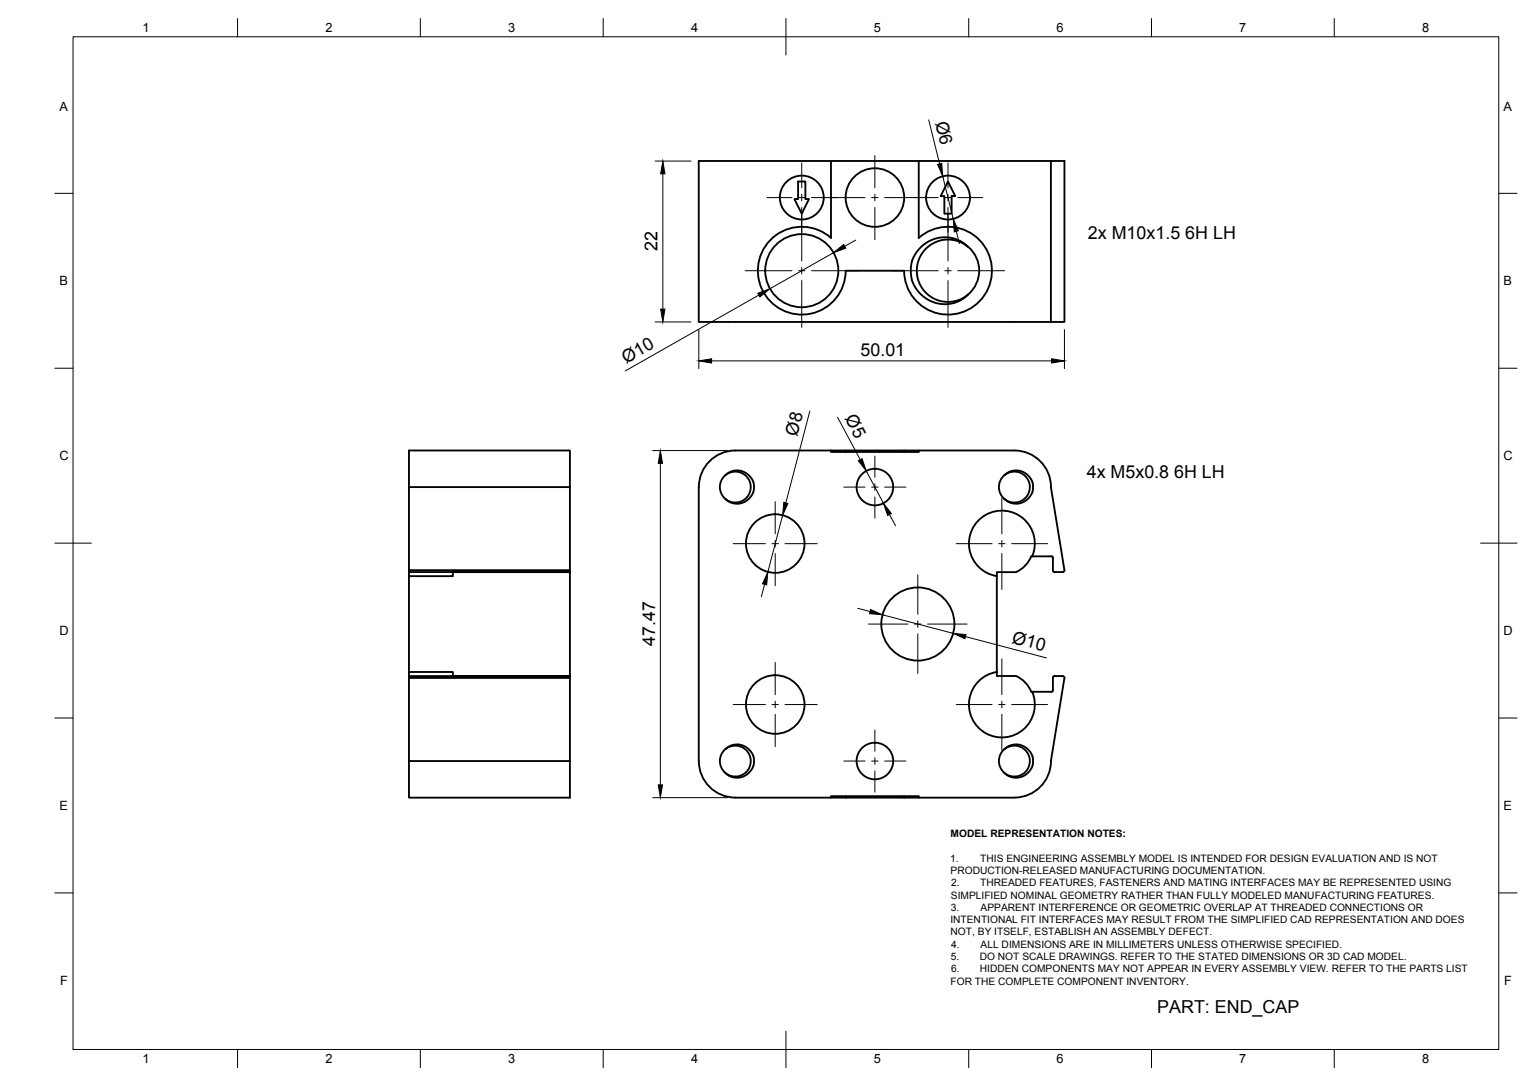
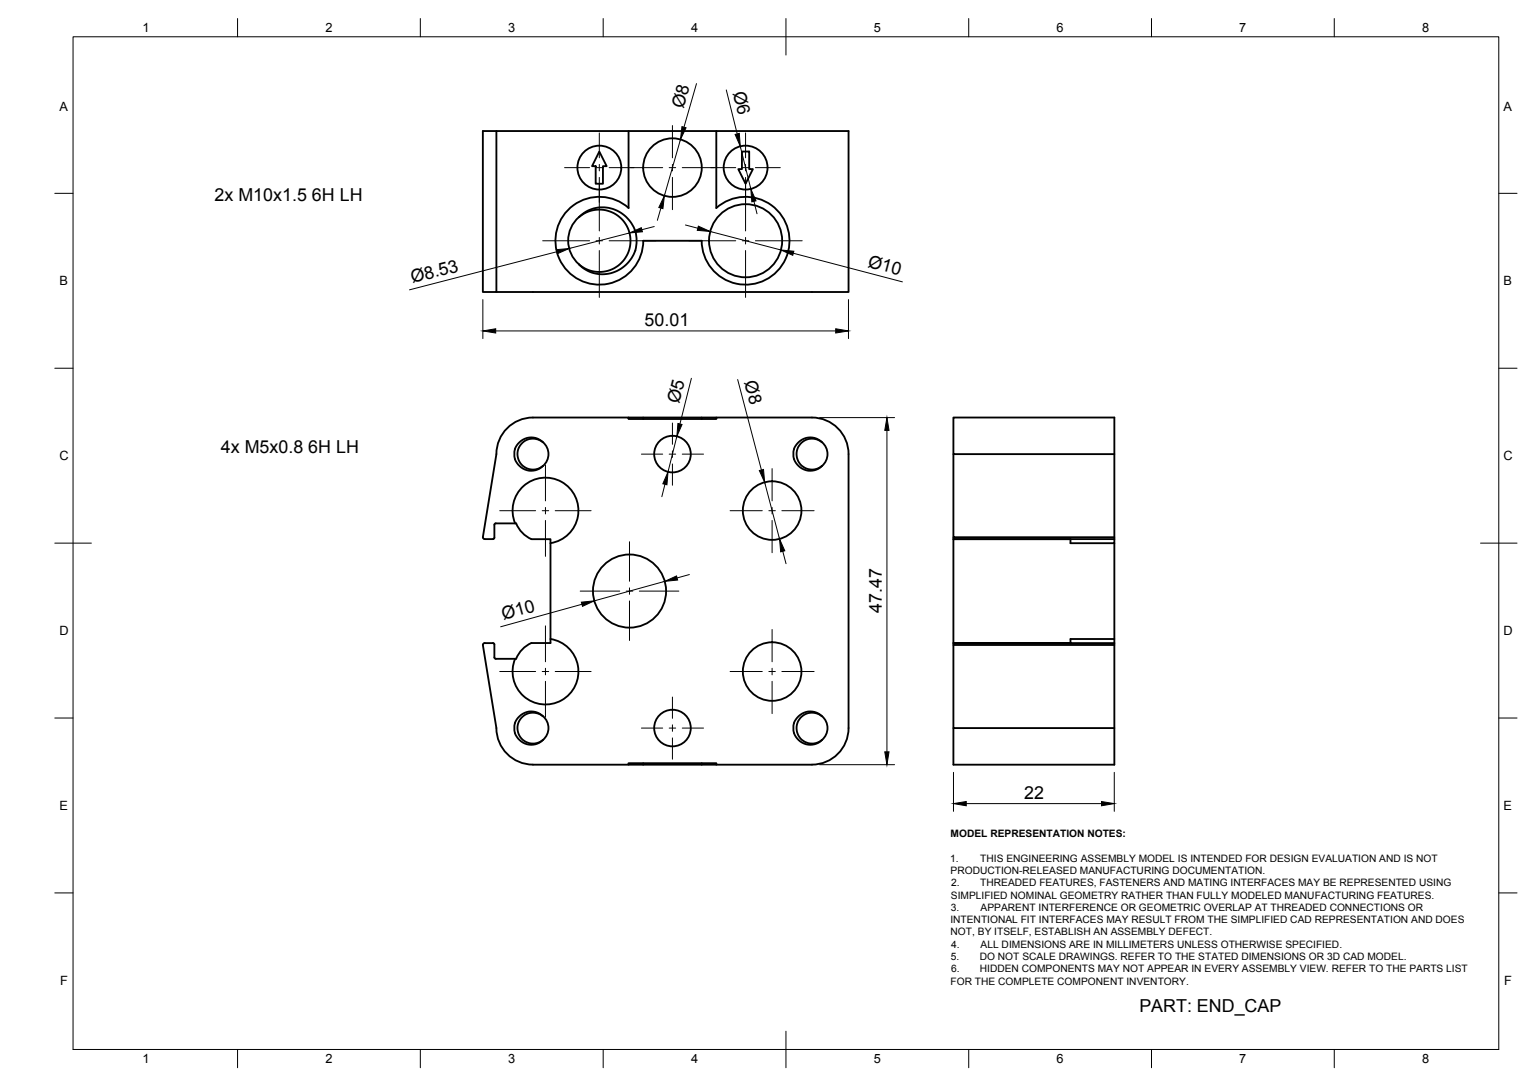
ISO-10303-21;
HEADER;
/* Generated by software containing ST-Developer
 * from STEP Tools, Inc. (www.steptools.com) 
 */

FILE_DESCRIPTION(
/* description */ (''),
/* implementation_level */ '2;1');

FILE_NAME(
/* name */ 'End_Cap.step',
/* time_stamp */ '2026-10-05T11:01:41-07:00',
/* author */ (''),
/* organization */ (''),
/* preprocessor_version */ 'ST-DEVELOPER v20.2',
/* originating_system */ 'Autodesk Translation Framework v15.15.0.0',
/* authorisation */ '');

FILE_SCHEMA (('AUTOMOTIVE_DESIGN { 1 0 10303 214 3 1 1 }'));
ENDSEC;

DATA;
#10=MECHANICAL_DESIGN_GEOMETRIC_PRESENTATION_REPRESENTATION('',(#2139),#215609);
#149=B_SPLINE_SURFACE_WITH_KNOTS('',3,3,((#115948,#115949,#115950,#115951,
#115952,#115953,#115954,#115955,#115956,#115957,#115958,#115959,#115960,
#115961,#115962,#115963,#115964,#115965,#115966,#115967,#115968,#115969,
#115970,#115971,#115972,#115973,#115974,#115975,#115976,#115977,#115978,
#115979,#115980,#115981,#115982,#115983,#115984,#115985,#115986,#115987,
#115988,#115989,#115990,#115991,#115992,#115993,#115994,#115995,#115996,
#115997,#115998,#115999,#116000,#116001),(#116002,#116003,#116004,#116005,
#116006,#116007,#116008,#116009,#116010,#116011,#116012,#116013,#116014,
#116015,#116016,#116017,#116018,#116019,#116020,#116021,#116022,#116023,
#116024,#116025,#116026,#116027,#116028,#116029,#116030,#116031,#116032,
#116033,#116034,#116035,#116036,#116037,#116038,#116039,#116040,#116041,
#116042,#116043,#116044,#116045,#116046,#116047,#116048,#116049,#116050,
#116051,#116052,#116053,#116054,#116055),(#116056,#116057,#116058,#116059,
#116060,#116061,#116062,#116063,#116064,#116065,#116066,#116067,#116068,
#116069,#116070,#116071,#116072,#116073,#116074,#116075,#116076,#116077,
#116078,#116079,#116080,#116081,#116082,#116083,#116084,#116085,#116086,
#116087,#116088,#116089,#116090,#116091,#116092,#116093,#116094,#116095,
#116096,#116097,#116098,#116099,#116100,#116101,#116102,#116103,#116104,
#116105,#116106,#116107,#116108,#116109),(#116110,#116111,#116112,#116113,
#116114,#116115,#116116,#116117,#116118,#116119,#116120,#116121,#116122,
#116123,#116124,#116125,#116126,#116127,#116128,#116129,#116130,#116131,
#116132,#116133,#116134,#116135,#116136,#116137,#116138,#116139,#116140,
#116141,#116142,#116143,#116144,#116145,#116146,#116147,#116148,#116149,
#116150,#116151,#116152,#116153,#116154,#116155,#116156,#116157,#116158,
#116159,#116160,#116161,#116162,#116163)),.UNSPECIFIED.,.F.,.F.,.F.,(4,
4),(4,1,1,1,1,1,1,1,1,1,1,1,1,1,1,1,1,1,1,1,1,1,1,1,1,1,1,1,1,1,1,1,1,1,
1,1,1,1,1,1,1,1,1,1,1,1,1,1,1,1,1,4),(-0.000626221895392836,0.0969365212249631),
(11.8528940954716,12.340290362188,12.8276378599491,13.3149853577101,13.8023328554711,
14.2896803532321,14.7770278509931,15.2643753487541,15.7517228465151,16.2390703442761,
16.7264178420371,17.2137653397981,17.7011128375591,18.1884603353201,18.6758078330811,
19.1631553308421,19.6505028286031,20.1378503263641,20.6251978241251,21.1125453218861,
21.5998928196471,22.0872403174081,22.5745878151691,23.0619353129301,23.5492828106911,
24.5239778062131,25.4986728017351,26.4733677972571,26.9607152950181,27.4480627927791,
27.9354102905401,28.4227577883011,28.9101052860621,29.3974527838231,29.8848002815841,
30.3721477793451,30.8594952771061,31.3468427748671,31.8341902726282,32.3215377703892,
32.8088852681502,33.2962327659112,33.7835802636722,34.2709277614332,34.7582752591942,
35.2456227569552,35.7329702547162,36.2203177524772,36.7076652502382,37.1950127479992,
37.6823602457602,38.1697077435212),.UNSPECIFIED.);
#150=B_SPLINE_SURFACE_WITH_KNOTS('',3,3,((#116370,#116371,#116372,#116373,
#116374,#116375,#116376,#116377,#116378,#116379,#116380,#116381,#116382,
#116383,#116384,#116385,#116386,#116387,#116388,#116389,#116390,#116391,
#116392,#116393,#116394,#116395,#116396,#116397,#116398,#116399,#116400,
#116401,#116402,#116403,#116404,#116405,#116406,#116407,#116408,#116409,
#116410,#116411,#116412,#116413,#116414,#116415,#116416,#116417,#116418,
#116419,#116420,#116421,#116422,#116423),(#116424,#116425,#116426,#116427,
#116428,#116429,#116430,#116431,#116432,#116433,#116434,#116435,#116436,
#116437,#116438,#116439,#116440,#116441,#116442,#116443,#116444,#116445,
#116446,#116447,#116448,#116449,#116450,#116451,#116452,#116453,#116454,
#116455,#116456,#116457,#116458,#116459,#116460,#116461,#116462,#116463,
#116464,#116465,#116466,#116467,#116468,#116469,#116470,#116471,#116472,
#116473,#116474,#116475,#116476,#116477),(#116478,#116479,#116480,#116481,
#116482,#116483,#116484,#116485,#116486,#116487,#116488,#116489,#116490,
#116491,#116492,#116493,#116494,#116495,#116496,#116497,#116498,#116499,
#116500,#116501,#116502,#116503,#116504,#116505,#116506,#116507,#116508,
#116509,#116510,#116511,#116512,#116513,#116514,#116515,#116516,#116517,
#116518,#116519,#116520,#116521,#116522,#116523,#116524,#116525,#116526,
#116527,#116528,#116529,#116530,#116531),(#116532,#116533,#116534,#116535,
#116536,#116537,#116538,#116539,#116540,#116541,#116542,#116543,#116544,
#116545,#116546,#116547,#116548,#116549,#116550,#116551,#116552,#116553,
#116554,#116555,#116556,#116557,#116558,#116559,#116560,#116561,#116562,
#116563,#116564,#116565,#116566,#116567,#116568,#116569,#116570,#116571,
#116572,#116573,#116574,#116575,#116576,#116577,#116578,#116579,#116580,
#116581,#116582,#116583,#116584,#116585)),.UNSPECIFIED.,.F.,.F.,.F.,(4,
4),(4,1,1,1,1,1,1,1,1,1,1,1,1,1,1,1,1,1,1,1,1,1,1,1,1,1,1,1,1,1,1,1,1,1,
1,1,1,1,1,1,1,1,1,1,1,1,1,1,1,1,1,4),(-0.000403511276840155,0.0967757900741628),
(14.399609326548,14.886956824309,15.37430432207,15.861651819831,16.348999317592,
16.836346815353,17.323694313114,17.811041810875,18.298389308636,18.785736806397,
19.273084304158,19.7604318019191,20.2477792996801,20.7351267974411,21.2224742952021,
21.7098217929631,22.1971692907241,22.6845167884851,23.1718642862461,23.6592117840071,
24.1465592817681,24.6339067795291,25.1212542772901,25.6086017750511,26.0959492728121,
27.0706442683341,28.0453392638561,29.0200342593781,29.5073817571391,29.9947292549001,
30.4820767526611,30.9694242504221,31.4567717481831,31.9441192459441,32.4314667437051,
32.9188142414661,33.4061617392271,33.8935092369881,34.3808567347491,34.8682042325101,
35.3555517302711,35.8428992280321,36.3302467257931,36.8175942235541,37.3049417213151,
37.7922892190762,38.2796367168372,38.7669842145982,39.2543317123592,39.7416792101202,
40.2290267078812,40.7164229770097),.UNSPECIFIED.);
#151=B_SPLINE_SURFACE_WITH_KNOTS('',3,3,((#116789,#116790,#116791,#116792,
#116793,#116794,#116795,#116796,#116797,#116798,#116799,#116800,#116801,
#116802,#116803,#116804,#116805,#116806,#116807,#116808,#116809,#116810,
#116811,#116812,#116813,#116814,#116815,#116816,#116817,#116818,#116819,
#116820,#116821,#116822,#116823,#116824,#116825,#116826,#116827,#116828,
#116829,#116830,#116831,#116832,#116833,#116834,#116835,#116836,#116837,
#116838,#116839,#116840,#116841,#116842),(#116843,#116844,#116845,#116846,
#116847,#116848,#116849,#116850,#116851,#116852,#116853,#116854,#116855,
#116856,#116857,#116858,#116859,#116860,#116861,#116862,#116863,#116864,
#116865,#116866,#116867,#116868,#116869,#116870,#116871,#116872,#116873,
#116874,#116875,#116876,#116877,#116878,#116879,#116880,#116881,#116882,
#116883,#116884,#116885,#116886,#116887,#116888,#116889,#116890,#116891,
#116892,#116893,#116894,#116895,#116896),(#116897,#116898,#116899,#116900,
#116901,#116902,#116903,#116904,#116905,#116906,#116907,#116908,#116909,
#116910,#116911,#116912,#116913,#116914,#116915,#116916,#116917,#116918,
#116919,#116920,#116921,#116922,#116923,#116924,#116925,#116926,#116927,
#116928,#116929,#116930,#116931,#116932,#116933,#116934,#116935,#116936,
#116937,#116938,#116939,#116940,#116941,#116942,#116943,#116944,#116945,
#116946,#116947,#116948,#116949,#116950),(#116951,#116952,#116953,#116954,
#116955,#116956,#116957,#116958,#116959,#116960,#116961,#116962,#116963,
#116964,#116965,#116966,#116967,#116968,#116969,#116970,#116971,#116972,
#116973,#116974,#116975,#116976,#116977,#116978,#116979,#116980,#116981,
#116982,#116983,#116984,#116985,#116986,#116987,#116988,#116989,#116990,
#116991,#116992,#116993,#116994,#116995,#116996,#116997,#116998,#116999,
#117000,#117001,#117002,#117003,#117004)),.UNSPECIFIED.,.F.,.F.,.F.,(4,
4),(4,1,1,1,1,1,1,1,1,1,1,1,1,1,1,1,1,1,1,1,1,1,1,1,1,1,1,1,1,1,1,1,1,1,
1,1,1,1,1,1,1,1,1,1,1,1,1,1,1,1,1,4),(-0.000626380093345518,0.0969365193294648),
(11.8528940858174,12.340290362188,12.827637859949,13.31498535771,13.802332855471,
14.289680353232,14.777027850993,15.264375348754,15.751722846515,16.239070344276,
16.7264178420371,17.2137653397981,17.7011128375591,18.1884603353201,18.6758078330811,
19.1631553308421,19.6505028286031,20.1378503263641,20.6251978241251,21.1125453218861,
21.5998928196471,22.0872403174081,22.5745878151691,23.0619353129301,23.5492828106911,
24.5239778062131,25.4986728017351,26.4733677972571,26.9607152950181,27.4480627927791,
27.9354102905401,28.4227577883011,28.9101052860621,29.3974527838231,29.8848002815841,
30.3721477793451,30.8594952771061,31.3468427748671,31.8341902726281,32.3215377703891,
32.8088852681501,33.2962327659111,33.7835802636721,34.2709277614331,34.7582752591941,
35.2456227569552,35.7329702547162,36.2203177524772,36.7076652502382,37.1950127479992,
37.6823602457602,38.1697077435212),.UNSPECIFIED.);
#152=B_SPLINE_SURFACE_WITH_KNOTS('',3,3,((#117214,#117215,#117216,#117217,
#117218,#117219,#117220,#117221,#117222,#117223,#117224,#117225,#117226,
#117227,#117228,#117229,#117230,#117231,#117232,#117233,#117234,#117235,
#117236,#117237,#117238,#117239,#117240,#117241,#117242,#117243,#117244,
#117245,#117246,#117247,#117248,#117249,#117250,#117251,#117252,#117253,
#117254,#117255,#117256,#117257,#117258,#117259,#117260,#117261,#117262,
#117263,#117264,#117265,#117266,#117267),(#117268,#117269,#117270,#117271,
#117272,#117273,#117274,#117275,#117276,#117277,#117278,#117279,#117280,
#117281,#117282,#117283,#117284,#117285,#117286,#117287,#117288,#117289,
#117290,#117291,#117292,#117293,#117294,#117295,#117296,#117297,#117298,
#117299,#117300,#117301,#117302,#117303,#117304,#117305,#117306,#117307,
#117308,#117309,#117310,#117311,#117312,#117313,#117314,#117315,#117316,
#117317,#117318,#117319,#117320,#117321),(#117322,#117323,#117324,#117325,
#117326,#117327,#117328,#117329,#117330,#117331,#117332,#117333,#117334,
#117335,#117336,#117337,#117338,#117339,#117340,#117341,#117342,#117343,
#117344,#117345,#117346,#117347,#117348,#117349,#117350,#117351,#117352,
#117353,#117354,#117355,#117356,#117357,#117358,#117359,#117360,#117361,
#117362,#117363,#117364,#117365,#117366,#117367,#117368,#117369,#117370,
#117371,#117372,#117373,#117374,#117375),(#117376,#117377,#117378,#117379,
#117380,#117381,#117382,#117383,#117384,#117385,#117386,#117387,#117388,
#117389,#117390,#117391,#117392,#117393,#117394,#117395,#117396,#117397,
#117398,#117399,#117400,#117401,#117402,#117403,#117404,#117405,#117406,
#117407,#117408,#117409,#117410,#117411,#117412,#117413,#117414,#117415,
#117416,#117417,#117418,#117419,#117420,#117421,#117422,#117423,#117424,
#117425,#117426,#117427,#117428,#117429)),.UNSPECIFIED.,.F.,.F.,.F.,(4,
4),(4,1,1,1,1,1,1,1,1,1,1,1,1,1,1,1,1,1,1,1,1,1,1,1,1,1,1,1,1,1,1,1,1,1,
1,1,1,1,1,1,1,1,1,1,1,1,1,1,1,1,1,4),(-0.000403508817394493,0.0967757699182735),
(14.399609326548,14.886956824309,15.37430432207,15.861651819831,16.348999317592,
16.836346815353,17.323694313114,17.811041810875,18.298389308636,18.785736806397,
19.273084304158,19.760431801919,20.24777929968,20.735126797441,21.222474295202,
21.709821792963,22.1971692907241,22.6845167884851,23.1718642862461,23.6592117840071,
24.1465592817681,24.6339067795291,25.1212542772901,25.6086017750511,26.0959492728121,
27.0706442683341,28.0453392638561,29.0200342593781,29.5073817571391,29.9947292549001,
30.4820767526611,30.9694242504221,31.4567717481831,31.9441192459441,32.4314667437051,
32.9188142414661,33.4061617392271,33.8935092369881,34.3808567347491,34.8682042325101,
35.3555517302711,35.8428992280321,36.3302467257931,36.8175942235541,37.3049417213151,
37.7922892190761,38.2796367168371,38.7669842145981,39.2543317123591,39.7416792101202,
40.2290267078812,40.7164229892059),.UNSPECIFIED.);
#153=B_SPLINE_SURFACE_WITH_KNOTS('',3,3,((#117642,#117643,#117644,#117645,
#117646,#117647,#117648,#117649,#117650,#117651,#117652,#117653,#117654,
#117655,#117656,#117657,#117658,#117659,#117660,#117661,#117662,#117663,
#117664,#117665,#117666,#117667,#117668,#117669,#117670,#117671,#117672,
#117673,#117674,#117675,#117676,#117677,#117678,#117679,#117680,#117681,
#117682,#117683,#117684,#117685,#117686,#117687,#117688,#117689,#117690,
#117691,#117692,#117693,#117694,#117695,#117696,#117697,#117698,#117699,
#117700,#117701,#117702,#117703,#117704,#117705,#117706,#117707,#117708,
#117709,#117710,#117711,#117712,#117713,#117714,#117715,#117716,#117717,
#117718,#117719,#117720,#117721,#117722,#117723,#117724,#117725,#117726,
#117727,#117728,#117729,#117730,#117731,#117732,#117733,#117734,#117735,
#117736,#117737,#117738,#117739,#117740,#117741,#117742,#117743,#117744,
#117745,#117746,#117747,#117748,#117749,#117750,#117751,#117752,#117753,
#117754,#117755,#117756,#117757,#117758,#117759,#117760,#117761,#117762,
#117763,#117764,#117765,#117766,#117767,#117768,#117769,#117770,#117771,
#117772,#117773,#117774,#117775,#117776,#117777,#117778,#117779,#117780,
#117781,#117782,#117783,#117784,#117785,#117786,#117787,#117788,#117789,
#117790,#117791,#117792,#117793,#117794,#117795,#117796,#117797,#117798,
#117799,#117800,#117801,#117802,#117803,#117804,#117805,#117806,#117807,
#117808,#117809,#117810,#117811,#117812,#117813,#117814,#117815,#117816,
#117817,#117818,#117819),(#117820,#117821,#117822,#117823,#117824,#117825,
#117826,#117827,#117828,#117829,#117830,#117831,#117832,#117833,#117834,
#117835,#117836,#117837,#117838,#117839,#117840,#117841,#117842,#117843,
#117844,#117845,#117846,#117847,#117848,#117849,#117850,#117851,#117852,
#117853,#117854,#117855,#117856,#117857,#117858,#117859,#117860,#117861,
#117862,#117863,#117864,#117865,#117866,#117867,#117868,#117869,#117870,
#117871,#117872,#117873,#117874,#117875,#117876,#117877,#117878,#117879,
#117880,#117881,#117882,#117883,#117884,#117885,#117886,#117887,#117888,
#117889,#117890,#117891,#117892,#117893,#117894,#117895,#117896,#117897,
#117898,#117899,#117900,#117901,#117902,#117903,#117904,#117905,#117906,
#117907,#117908,#117909,#117910,#117911,#117912,#117913,#117914,#117915,
#117916,#117917,#117918,#117919,#117920,#117921,#117922,#117923,#117924,
#117925,#117926,#117927,#117928,#117929,#117930,#117931,#117932,#117933,
#117934,#117935,#117936,#117937,#117938,#117939,#117940,#117941,#117942,
#117943,#117944,#117945,#117946,#117947,#117948,#117949,#117950,#117951,
#117952,#117953,#117954,#117955,#117956,#117957,#117958,#117959,#117960,
#117961,#117962,#117963,#117964,#117965,#117966,#117967,#117968,#117969,
#117970,#117971,#117972,#117973,#117974,#117975,#117976,#117977,#117978,
#117979,#117980,#117981,#117982,#117983,#117984,#117985,#117986,#117987,
#117988,#117989,#117990,#117991,#117992,#117993,#117994,#117995,#117996,
#117997),(#117998,#117999,#118000,#118001,#118002,#118003,#118004,#118005,
#118006,#118007,#118008,#118009,#118010,#118011,#118012,#118013,#118014,
#118015,#118016,#118017,#118018,#118019,#118020,#118021,#118022,#118023,
#118024,#118025,#118026,#118027,#118028,#118029,#118030,#118031,#118032,
#118033,#118034,#118035,#118036,#118037,#118038,#118039,#118040,#118041,
#118042,#118043,#118044,#118045,#118046,#118047,#118048,#118049,#118050,
#118051,#118052,#118053,#118054,#118055,#118056,#118057,#118058,#118059,
#118060,#118061,#118062,#118063,#118064,#118065,#118066,#118067,#118068,
#118069,#118070,#118071,#118072,#118073,#118074,#118075,#118076,#118077,
#118078,#118079,#118080,#118081,#118082,#118083,#118084,#118085,#118086,
#118087,#118088,#118089,#118090,#118091,#118092,#118093,#118094,#118095,
#118096,#118097,#118098,#118099,#118100,#118101,#118102,#118103,#118104,
#118105,#118106,#118107,#118108,#118109,#118110,#118111,#118112,#118113,
#118114,#118115,#118116,#118117,#118118,#118119,#118120,#118121,#118122,
#118123,#118124,#118125,#118126,#118127,#118128,#118129,#118130,#118131,
#118132,#118133,#118134,#118135,#118136,#118137,#118138,#118139,#118140,
#118141,#118142,#118143,#118144,#118145,#118146,#118147,#118148,#118149,
#118150,#118151,#118152,#118153,#118154,#118155,#118156,#118157,#118158,
#118159,#118160,#118161,#118162,#118163,#118164,#118165,#118166,#118167,
#118168,#118169,#118170,#118171,#118172,#118173,#118174,#118175),(#118176,
#118177,#118178,#118179,#118180,#118181,#118182,#118183,#118184,#118185,
#118186,#118187,#118188,#118189,#118190,#118191,#118192,#118193,#118194,
#118195,#118196,#118197,#118198,#118199,#118200,#118201,#118202,#118203,
#118204,#118205,#118206,#118207,#118208,#118209,#118210,#118211,#118212,
#118213,#118214,#118215,#118216,#118217,#118218,#118219,#118220,#118221,
#118222,#118223,#118224,#118225,#118226,#118227,#118228,#118229,#118230,
#118231,#118232,#118233,#118234,#118235,#118236,#118237,#118238,#118239,
#118240,#118241,#118242,#118243,#118244,#118245,#118246,#118247,#118248,
#118249,#118250,#118251,#118252,#118253,#118254,#118255,#118256,#118257,
#118258,#118259,#118260,#118261,#118262,#118263,#118264,#118265,#118266,
#118267,#118268,#118269,#118270,#118271,#118272,#118273,#118274,#118275,
#118276,#118277,#118278,#118279,#118280,#118281,#118282,#118283,#118284,
#118285,#118286,#118287,#118288,#118289,#118290,#118291,#118292,#118293,
#118294,#118295,#118296,#118297,#118298,#118299,#118300,#118301,#118302,
#118303,#118304,#118305,#118306,#118307,#118308,#118309,#118310,#118311,
#118312,#118313,#118314,#118315,#118316,#118317,#118318,#118319,#118320,
#118321,#118322,#118323,#118324,#118325,#118326,#118327,#118328,#118329,
#118330,#118331,#118332,#118333,#118334,#118335,#118336,#118337,#118338,
#118339,#118340,#118341,#118342,#118343,#118344,#118345,#118346,#118347,
#118348,#118349,#118350,#118351,#118352,#118353)),.UNSPECIFIED.,.F.,.F.,
 .F.,(4,4),(4,1,1,1,1,1,1,1,1,1,1,1,1,1,1,1,1,1,1,1,1,1,1,1,1,1,1,1,1,1,
1,1,1,1,1,1,1,1,1,1,1,1,1,1,1,1,1,1,1,1,1,1,1,1,1,1,1,1,1,1,1,1,1,1,1,1,
1,1,1,1,1,1,1,1,1,1,1,1,1,1,1,1,1,1,1,1,1,1,1,1,1,1,1,1,1,1,1,1,1,1,1,1,
1,1,1,1,1,1,1,1,1,1,1,1,1,1,1,1,1,1,1,1,1,1,1,1,1,1,1,1,1,1,1,1,1,1,1,1,
1,1,1,1,1,1,1,1,1,1,1,1,1,1,1,1,1,1,1,1,1,1,1,1,1,1,1,1,1,1,1,1,1,1,1,1,
1,4),(-0.000439606948779746,0.0515314320759051),(11.8664846275776,12.8657606844883,
13.8645971344502,14.8634335844121,15.8622700343739,16.8611064843358,17.8599429342977,
18.8587793842595,19.8576158342214,20.8564522841833,21.8552887341452,22.854125184107,
23.8529616340689,24.8517980840308,25.8506345339927,26.8494709839545,27.8483074339164,
28.8471438838783,29.8459803338402,30.844816783802,31.8436532337639,32.8424896837258,
33.8413261336877,34.8401625836495,35.8389990336114,36.8378354835733,37.8366719335352,
38.835508383497,39.8343448334589,40.8331812834208,41.8320177333826,42.8308541833445,
43.8296906333064,44.8285270832683,45.8273635332301,46.826199983192,47.8250364331539,
48.8238728831158,49.8227093330776,50.8215457830395,51.8203822330014,52.8192186829633,
53.8180551329251,54.816891582887,55.8157280328489,56.8145644828108,57.8134009327726,
58.8122373827345,59.8110738326964,60.8099102826583,61.8087467326201,62.807583182582,
63.8064196325439,64.8052560825058,65.8040925324676,66.8029289824295,67.8017654323914,
68.8006018823532,69.7994383323151,70.798274782277,71.7971112322389,72.7959476822007,
73.7947841321626,74.7936205821245,75.7924570320864,76.7912934820482,77.7901299320101,
78.788966381972,79.7878028319339,80.7866392818957,81.7854757318576,82.7843121818195,
83.7831486317814,84.7819850817432,85.7808215317051,86.779657981667,87.7784944316288,
88.7773308815907,89.7761673315526,90.7750037815145,91.7738402314764,92.7726766814382,
93.7715131314001,94.770349581362,95.7691860313238,96.7680224812857,97.7668589312476,
98.7656953812095,99.7645318311714,100.763368281133,101.762204731095,102.761041181057,
103.759877631019,104.758714080981,105.757550530943,106.756386980904,107.755223430866,
108.754059880828,109.75289633079,110.751732780752,111.750569230714,112.749405680676,
113.748242130638,114.747078580599,115.745915030561,116.744751480523,117.743587930485,
118.742424380447,119.741260830409,120.740097280371,121.738933730333,122.737770180294,
123.736606630256,124.735443080218,125.73427953018,126.733115980142,127.731952430104,
128.730788880066,129.729625330028,130.728461779989,131.727298229951,132.726134679913,
133.724971129875,134.723807579837,135.722644029799,136.721480479761,137.720316929723,
138.719153379684,139.717989829646,140.716826279608,141.71566272957,142.714499179532,
143.713335629494,144.712172079456,145.711008529418,146.709844979379,147.708681429341,
148.707517879303,149.706354329265,150.705190779227,151.704027229189,152.702863679151,
153.701700129113,154.700536579074,155.699373029036,156.698209478998,157.69704592896,
158.695882378922,159.694718828884,160.693555278846,161.692391728808,162.691228178769,
163.690064628731,164.688901078693,165.687737528655,166.686573978617,167.685410428579,
168.684246878541,169.683083328503,170.681919778464,171.680756228426,172.679592678388,
173.67842912835,174.677265578312,175.676102028274,176.674938478236,177.673774928198,
178.672611378159,179.671447828121,180.670284278083,181.669120728045,182.667957178007,
183.666793627969,184.665630077931,185.664466527893,186.663302977854),
 .UNSPECIFIED.);
#154=B_SPLINE_SURFACE_WITH_KNOTS('',3,3,((#118442,#118443,#118444,#118445,
#118446,#118447,#118448,#118449,#118450,#118451,#118452,#118453,#118454,
#118455,#118456,#118457,#118458,#118459,#118460,#118461,#118462,#118463,
#118464,#118465,#118466,#118467,#118468,#118469,#118470,#118471,#118472,
#118473,#118474,#118475,#118476,#118477,#118478,#118479,#118480,#118481,
#118482,#118483,#118484,#118485,#118486,#118487,#118488,#118489,#118490,
#118491,#118492,#118493,#118494,#118495,#118496,#118497,#118498,#118499,
#118500,#118501,#118502,#118503,#118504,#118505,#118506,#118507,#118508,
#118509,#118510,#118511,#118512,#118513,#118514,#118515,#118516,#118517,
#118518,#118519,#118520,#118521,#118522,#118523,#118524,#118525,#118526,
#118527,#118528,#118529,#118530,#118531,#118532,#118533,#118534,#118535,
#118536,#118537,#118538,#118539,#118540,#118541,#118542,#118543,#118544,
#118545,#118546,#118547,#118548,#118549,#118550,#118551,#118552,#118553,
#118554,#118555,#118556,#118557,#118558,#118559,#118560,#118561,#118562,
#118563,#118564,#118565,#118566,#118567,#118568,#118569,#118570,#118571,
#118572,#118573,#118574,#118575,#118576,#118577,#118578,#118579,#118580,
#118581,#118582,#118583,#118584,#118585,#118586,#118587,#118588,#118589,
#118590,#118591,#118592,#118593,#118594,#118595,#118596,#118597,#118598,
#118599,#118600,#118601,#118602,#118603,#118604,#118605,#118606,#118607,
#118608,#118609,#118610,#118611,#118612,#118613,#118614,#118615,#118616,
#118617,#118618,#118619),(#118620,#118621,#118622,#118623,#118624,#118625,
#118626,#118627,#118628,#118629,#118630,#118631,#118632,#118633,#118634,
#118635,#118636,#118637,#118638,#118639,#118640,#118641,#118642,#118643,
#118644,#118645,#118646,#118647,#118648,#118649,#118650,#118651,#118652,
#118653,#118654,#118655,#118656,#118657,#118658,#118659,#118660,#118661,
#118662,#118663,#118664,#118665,#118666,#118667,#118668,#118669,#118670,
#118671,#118672,#118673,#118674,#118675,#118676,#118677,#118678,#118679,
#118680,#118681,#118682,#118683,#118684,#118685,#118686,#118687,#118688,
#118689,#118690,#118691,#118692,#118693,#118694,#118695,#118696,#118697,
#118698,#118699,#118700,#118701,#118702,#118703,#118704,#118705,#118706,
#118707,#118708,#118709,#118710,#118711,#118712,#118713,#118714,#118715,
#118716,#118717,#118718,#118719,#118720,#118721,#118722,#118723,#118724,
#118725,#118726,#118727,#118728,#118729,#118730,#118731,#118732,#118733,
#118734,#118735,#118736,#118737,#118738,#118739,#118740,#118741,#118742,
#118743,#118744,#118745,#118746,#118747,#118748,#118749,#118750,#118751,
#118752,#118753,#118754,#118755,#118756,#118757,#118758,#118759,#118760,
#118761,#118762,#118763,#118764,#118765,#118766,#118767,#118768,#118769,
#118770,#118771,#118772,#118773,#118774,#118775,#118776,#118777,#118778,
#118779,#118780,#118781,#118782,#118783,#118784,#118785,#118786,#118787,
#118788,#118789,#118790,#118791,#118792,#118793,#118794,#118795,#118796,
#118797),(#118798,#118799,#118800,#118801,#118802,#118803,#118804,#118805,
#118806,#118807,#118808,#118809,#118810,#118811,#118812,#118813,#118814,
#118815,#118816,#118817,#118818,#118819,#118820,#118821,#118822,#118823,
#118824,#118825,#118826,#118827,#118828,#118829,#118830,#118831,#118832,
#118833,#118834,#118835,#118836,#118837,#118838,#118839,#118840,#118841,
#118842,#118843,#118844,#118845,#118846,#118847,#118848,#118849,#118850,
#118851,#118852,#118853,#118854,#118855,#118856,#118857,#118858,#118859,
#118860,#118861,#118862,#118863,#118864,#118865,#118866,#118867,#118868,
#118869,#118870,#118871,#118872,#118873,#118874,#118875,#118876,#118877,
#118878,#118879,#118880,#118881,#118882,#118883,#118884,#118885,#118886,
#118887,#118888,#118889,#118890,#118891,#118892,#118893,#118894,#118895,
#118896,#118897,#118898,#118899,#118900,#118901,#118902,#118903,#118904,
#118905,#118906,#118907,#118908,#118909,#118910,#118911,#118912,#118913,
#118914,#118915,#118916,#118917,#118918,#118919,#118920,#118921,#118922,
#118923,#118924,#118925,#118926,#118927,#118928,#118929,#118930,#118931,
#118932,#118933,#118934,#118935,#118936,#118937,#118938,#118939,#118940,
#118941,#118942,#118943,#118944,#118945,#118946,#118947,#118948,#118949,
#118950,#118951,#118952,#118953,#118954,#118955,#118956,#118957,#118958,
#118959,#118960,#118961,#118962,#118963,#118964,#118965,#118966,#118967,
#118968,#118969,#118970,#118971,#118972,#118973,#118974,#118975),(#118976,
#118977,#118978,#118979,#118980,#118981,#118982,#118983,#118984,#118985,
#118986,#118987,#118988,#118989,#118990,#118991,#118992,#118993,#118994,
#118995,#118996,#118997,#118998,#118999,#119000,#119001,#119002,#119003,
#119004,#119005,#119006,#119007,#119008,#119009,#119010,#119011,#119012,
#119013,#119014,#119015,#119016,#119017,#119018,#119019,#119020,#119021,
#119022,#119023,#119024,#119025,#119026,#119027,#119028,#119029,#119030,
#119031,#119032,#119033,#119034,#119035,#119036,#119037,#119038,#119039,
#119040,#119041,#119042,#119043,#119044,#119045,#119046,#119047,#119048,
#119049,#119050,#119051,#119052,#119053,#119054,#119055,#119056,#119057,
#119058,#119059,#119060,#119061,#119062,#119063,#119064,#119065,#119066,
#119067,#119068,#119069,#119070,#119071,#119072,#119073,#119074,#119075,
#119076,#119077,#119078,#119079,#119080,#119081,#119082,#119083,#119084,
#119085,#119086,#119087,#119088,#119089,#119090,#119091,#119092,#119093,
#119094,#119095,#119096,#119097,#119098,#119099,#119100,#119101,#119102,
#119103,#119104,#119105,#119106,#119107,#119108,#119109,#119110,#119111,
#119112,#119113,#119114,#119115,#119116,#119117,#119118,#119119,#119120,
#119121,#119122,#119123,#119124,#119125,#119126,#119127,#119128,#119129,
#119130,#119131,#119132,#119133,#119134,#119135,#119136,#119137,#119138,
#119139,#119140,#119141,#119142,#119143,#119144,#119145,#119146,#119147,
#119148,#119149,#119150,#119151,#119152,#119153)),.UNSPECIFIED.,.F.,.F.,
 .F.,(4,4),(4,1,1,1,1,1,1,1,1,1,1,1,1,1,1,1,1,1,1,1,1,1,1,1,1,1,1,1,1,1,
1,1,1,1,1,1,1,1,1,1,1,1,1,1,1,1,1,1,1,1,1,1,1,1,1,1,1,1,1,1,1,1,1,1,1,1,
1,1,1,1,1,1,1,1,1,1,1,1,1,1,1,1,1,1,1,1,1,1,1,1,1,1,1,1,1,1,1,1,1,1,1,1,
1,1,1,1,1,1,1,1,1,1,1,1,1,1,1,1,1,1,1,1,1,1,1,1,1,1,1,1,1,1,1,1,1,1,1,1,
1,1,1,1,1,1,1,1,1,1,1,1,1,1,1,1,1,1,1,1,1,1,1,1,1,1,1,1,1,1,1,1,1,1,1,1,
1,4),(-0.000378201108639058,0.051592837406338),(14.3986268518925,15.3974633018543,
16.3962997518162,17.3951362017781,18.39397265174,19.3928091017018,20.3916455516637,
21.3904820016256,22.3893184515875,23.3881549015493,24.3869913515112,25.3858278014731,
26.3846642514349,27.3835007013968,28.3823371513587,29.3811736013206,30.3800100512824,
31.3788465012443,32.3776829512062,33.3765194011681,34.3753558511299,35.3741923010918,
36.3730287510537,37.3718652010156,38.3707016509774,39.3695381009393,40.3683745509012,
41.3672110008631,42.3660474508249,43.3648839007868,44.3637203507487,45.3625568007106,
46.3613932506724,47.3602297006343,48.3590661505962,49.3579026005581,50.3567390505199,
51.3555755004818,52.3544119504437,53.3532484004055,54.3520848503674,55.3509213003293,
56.3497577502912,57.348594200253,58.3474306502149,59.3462671001768,60.3451035501387,
61.3439400001005,62.3427764500624,63.3416129000243,64.3404493499862,65.339285799948,
66.3381222499099,67.3369586998718,68.3357951498337,69.3346315997955,70.3334680497574,
71.3323044997193,72.3311409496812,73.329977399643,74.3288138496049,75.3276502995668,
76.3264867495287,77.3253231994905,78.3241596494524,79.3229960994143,80.3218325493762,
81.320668999338,82.3195054492999,83.3183418992618,84.3171783492237,85.3160147991855,
86.3148512491474,87.3136876991093,88.3125241490712,89.311360599033,90.3101970489949,
91.3090334989568,92.3078699489186,93.3067063988805,94.3055428488424,95.3043792988043,
96.3032157487661,97.302052198728,98.3008886486899,99.2997250986518,100.298561548614,
101.297397998576,102.296234448537,103.295070898499,104.293907348461,105.292743798423,
106.291580248385,107.290416698347,108.289253148309,109.288089598271,110.286926048232,
111.285762498194,112.284598948156,113.283435398118,114.28227184808,115.281108298042,
116.279944748004,117.278781197966,118.277617647927,119.276454097889,120.275290547851,
121.274126997813,122.272963447775,123.271799897737,124.270636347699,125.26947279766,
126.268309247622,127.267145697584,128.265982147546,129.264818597508,130.26365504747,
131.262491497432,132.261327947394,133.260164397355,134.259000847317,135.257837297279,
136.256673747241,137.255510197203,138.254346647165,139.253183097127,140.252019547089,
141.25085599705,142.249692447012,143.248528896974,144.247365346936,145.246201796898,
146.24503824686,147.243874696822,148.242711146784,149.241547596745,150.240384046707,
151.239220496669,152.238056946631,153.236893396593,154.235729846555,155.234566296517,
156.233402746479,157.23223919644,158.231075646402,159.229912096364,160.228748546326,
161.227584996288,162.22642144625,163.225257896212,164.224094346174,165.222930796135,
166.221767246097,167.220603696059,168.219440146021,169.218276595983,170.217113045945,
171.215949495907,172.214785945869,173.21362239583,174.212458845792,175.211295295754,
176.210131745716,177.208968195678,178.20780464564,179.206641095602,180.205477545564,
181.204313995525,182.203150445487,183.201986895449,184.200823345411,185.199659795373,
186.198496245335,187.197332695297,188.196169145259,189.195445198776),
 .UNSPECIFIED.);
#155=B_SPLINE_SURFACE_WITH_KNOTS('',3,3,((#119245,#119246,#119247,#119248,
#119249,#119250,#119251,#119252,#119253,#119254,#119255,#119256,#119257,
#119258,#119259,#119260,#119261,#119262,#119263,#119264,#119265,#119266,
#119267,#119268,#119269,#119270,#119271,#119272,#119273,#119274,#119275,
#119276,#119277,#119278,#119279,#119280,#119281,#119282,#119283,#119284,
#119285,#119286,#119287,#119288,#119289,#119290,#119291,#119292,#119293,
#119294,#119295,#119296,#119297,#119298,#119299,#119300,#119301,#119302,
#119303,#119304,#119305,#119306,#119307,#119308,#119309,#119310,#119311,
#119312,#119313,#119314,#119315,#119316,#119317,#119318,#119319,#119320,
#119321,#119322,#119323,#119324,#119325,#119326,#119327,#119328,#119329,
#119330,#119331,#119332,#119333,#119334,#119335,#119336,#119337,#119338,
#119339,#119340,#119341,#119342,#119343,#119344,#119345,#119346,#119347,
#119348,#119349,#119350,#119351,#119352,#119353,#119354,#119355,#119356,
#119357,#119358,#119359,#119360,#119361,#119362,#119363,#119364,#119365,
#119366,#119367,#119368,#119369,#119370,#119371,#119372,#119373,#119374,
#119375,#119376,#119377,#119378,#119379,#119380,#119381,#119382,#119383,
#119384,#119385,#119386,#119387,#119388,#119389,#119390,#119391,#119392,
#119393,#119394,#119395,#119396,#119397,#119398,#119399,#119400,#119401,
#119402,#119403,#119404,#119405,#119406,#119407,#119408,#119409,#119410,
#119411,#119412,#119413,#119414,#119415,#119416,#119417,#119418,#119419,
#119420,#119421,#119422),(#119423,#119424,#119425,#119426,#119427,#119428,
#119429,#119430,#119431,#119432,#119433,#119434,#119435,#119436,#119437,
#119438,#119439,#119440,#119441,#119442,#119443,#119444,#119445,#119446,
#119447,#119448,#119449,#119450,#119451,#119452,#119453,#119454,#119455,
#119456,#119457,#119458,#119459,#119460,#119461,#119462,#119463,#119464,
#119465,#119466,#119467,#119468,#119469,#119470,#119471,#119472,#119473,
#119474,#119475,#119476,#119477,#119478,#119479,#119480,#119481,#119482,
#119483,#119484,#119485,#119486,#119487,#119488,#119489,#119490,#119491,
#119492,#119493,#119494,#119495,#119496,#119497,#119498,#119499,#119500,
#119501,#119502,#119503,#119504,#119505,#119506,#119507,#119508,#119509,
#119510,#119511,#119512,#119513,#119514,#119515,#119516,#119517,#119518,
#119519,#119520,#119521,#119522,#119523,#119524,#119525,#119526,#119527,
#119528,#119529,#119530,#119531,#119532,#119533,#119534,#119535,#119536,
#119537,#119538,#119539,#119540,#119541,#119542,#119543,#119544,#119545,
#119546,#119547,#119548,#119549,#119550,#119551,#119552,#119553,#119554,
#119555,#119556,#119557,#119558,#119559,#119560,#119561,#119562,#119563,
#119564,#119565,#119566,#119567,#119568,#119569,#119570,#119571,#119572,
#119573,#119574,#119575,#119576,#119577,#119578,#119579,#119580,#119581,
#119582,#119583,#119584,#119585,#119586,#119587,#119588,#119589,#119590,
#119591,#119592,#119593,#119594,#119595,#119596,#119597,#119598,#119599,
#119600),(#119601,#119602,#119603,#119604,#119605,#119606,#119607,#119608,
#119609,#119610,#119611,#119612,#119613,#119614,#119615,#119616,#119617,
#119618,#119619,#119620,#119621,#119622,#119623,#119624,#119625,#119626,
#119627,#119628,#119629,#119630,#119631,#119632,#119633,#119634,#119635,
#119636,#119637,#119638,#119639,#119640,#119641,#119642,#119643,#119644,
#119645,#119646,#119647,#119648,#119649,#119650,#119651,#119652,#119653,
#119654,#119655,#119656,#119657,#119658,#119659,#119660,#119661,#119662,
#119663,#119664,#119665,#119666,#119667,#119668,#119669,#119670,#119671,
#119672,#119673,#119674,#119675,#119676,#119677,#119678,#119679,#119680,
#119681,#119682,#119683,#119684,#119685,#119686,#119687,#119688,#119689,
#119690,#119691,#119692,#119693,#119694,#119695,#119696,#119697,#119698,
#119699,#119700,#119701,#119702,#119703,#119704,#119705,#119706,#119707,
#119708,#119709,#119710,#119711,#119712,#119713,#119714,#119715,#119716,
#119717,#119718,#119719,#119720,#119721,#119722,#119723,#119724,#119725,
#119726,#119727,#119728,#119729,#119730,#119731,#119732,#119733,#119734,
#119735,#119736,#119737,#119738,#119739,#119740,#119741,#119742,#119743,
#119744,#119745,#119746,#119747,#119748,#119749,#119750,#119751,#119752,
#119753,#119754,#119755,#119756,#119757,#119758,#119759,#119760,#119761,
#119762,#119763,#119764,#119765,#119766,#119767,#119768,#119769,#119770,
#119771,#119772,#119773,#119774,#119775,#119776,#119777,#119778),(#119779,
#119780,#119781,#119782,#119783,#119784,#119785,#119786,#119787,#119788,
#119789,#119790,#119791,#119792,#119793,#119794,#119795,#119796,#119797,
#119798,#119799,#119800,#119801,#119802,#119803,#119804,#119805,#119806,
#119807,#119808,#119809,#119810,#119811,#119812,#119813,#119814,#119815,
#119816,#119817,#119818,#119819,#119820,#119821,#119822,#119823,#119824,
#119825,#119826,#119827,#119828,#119829,#119830,#119831,#119832,#119833,
#119834,#119835,#119836,#119837,#119838,#119839,#119840,#119841,#119842,
#119843,#119844,#119845,#119846,#119847,#119848,#119849,#119850,#119851,
#119852,#119853,#119854,#119855,#119856,#119857,#119858,#119859,#119860,
#119861,#119862,#119863,#119864,#119865,#119866,#119867,#119868,#119869,
#119870,#119871,#119872,#119873,#119874,#119875,#119876,#119877,#119878,
#119879,#119880,#119881,#119882,#119883,#119884,#119885,#119886,#119887,
#119888,#119889,#119890,#119891,#119892,#119893,#119894,#119895,#119896,
#119897,#119898,#119899,#119900,#119901,#119902,#119903,#119904,#119905,
#119906,#119907,#119908,#119909,#119910,#119911,#119912,#119913,#119914,
#119915,#119916,#119917,#119918,#119919,#119920,#119921,#119922,#119923,
#119924,#119925,#119926,#119927,#119928,#119929,#119930,#119931,#119932,
#119933,#119934,#119935,#119936,#119937,#119938,#119939,#119940,#119941,
#119942,#119943,#119944,#119945,#119946,#119947,#119948,#119949,#119950,
#119951,#119952,#119953,#119954,#119955,#119956)),.UNSPECIFIED.,.F.,.F.,
 .F.,(4,4),(4,1,1,1,1,1,1,1,1,1,1,1,1,1,1,1,1,1,1,1,1,1,1,1,1,1,1,1,1,1,
1,1,1,1,1,1,1,1,1,1,1,1,1,1,1,1,1,1,1,1,1,1,1,1,1,1,1,1,1,1,1,1,1,1,1,1,
1,1,1,1,1,1,1,1,1,1,1,1,1,1,1,1,1,1,1,1,1,1,1,1,1,1,1,1,1,1,1,1,1,1,1,1,
1,1,1,1,1,1,1,1,1,1,1,1,1,1,1,1,1,1,1,1,1,1,1,1,1,1,1,1,1,1,1,1,1,1,1,1,
1,1,1,1,1,1,1,1,1,1,1,1,1,1,1,1,1,1,1,1,1,1,1,1,1,1,1,1,1,1,1,1,1,1,1,1,
1,4),(-0.000439572862182687,0.0515314610720387),(11.8664846616642,12.8657606844883,
13.8645971344502,14.8634335844121,15.8622700343739,16.8611064843358,17.8599429342977,
18.8587793842595,19.8576158342214,20.8564522841833,21.8552887341452,22.854125184107,
23.8529616340689,24.8517980840308,25.8506345339927,26.8494709839545,27.8483074339164,
28.8471438838783,29.8459803338402,30.844816783802,31.8436532337639,32.8424896837258,
33.8413261336877,34.8401625836495,35.8389990336114,36.8378354835733,37.8366719335352,
38.835508383497,39.8343448334589,40.8331812834208,41.8320177333826,42.8308541833445,
43.8296906333064,44.8285270832683,45.8273635332301,46.826199983192,47.8250364331539,
48.8238728831158,49.8227093330776,50.8215457830395,51.8203822330014,52.8192186829633,
53.8180551329251,54.816891582887,55.8157280328489,56.8145644828108,57.8134009327726,
58.8122373827345,59.8110738326964,60.8099102826583,61.8087467326201,62.807583182582,
63.8064196325439,64.8052560825058,65.8040925324676,66.8029289824295,67.8017654323914,
68.8006018823532,69.7994383323151,70.798274782277,71.7971112322389,72.7959476822007,
73.7947841321626,74.7936205821245,75.7924570320864,76.7912934820482,77.7901299320101,
78.788966381972,79.7878028319339,80.7866392818957,81.7854757318576,82.7843121818195,
83.7831486317814,84.7819850817432,85.7808215317051,86.779657981667,87.7784944316289,
88.7773308815907,89.7761673315526,90.7750037815145,91.7738402314764,92.7726766814382,
93.7715131314001,94.770349581362,95.7691860313239,96.7680224812857,97.7668589312476,
98.7656953812095,99.7645318311714,100.763368281133,101.762204731095,102.761041181057,
103.759877631019,104.758714080981,105.757550530943,106.756386980904,107.755223430866,
108.754059880828,109.75289633079,110.751732780752,111.750569230714,112.749405680676,
113.748242130638,114.747078580599,115.745915030561,116.744751480523,117.743587930485,
118.742424380447,119.741260830409,120.740097280371,121.738933730333,122.737770180294,
123.736606630256,124.735443080218,125.73427953018,126.733115980142,127.731952430104,
128.730788880066,129.729625330028,130.728461779989,131.727298229951,132.726134679913,
133.724971129875,134.723807579837,135.722644029799,136.721480479761,137.720316929723,
138.719153379684,139.717989829646,140.716826279608,141.71566272957,142.714499179532,
143.713335629494,144.712172079456,145.711008529418,146.709844979379,147.708681429341,
148.707517879303,149.706354329265,150.705190779227,151.704027229189,152.702863679151,
153.701700129113,154.700536579074,155.699373029036,156.698209478998,157.69704592896,
158.695882378922,159.694718828884,160.693555278846,161.692391728808,162.691228178769,
163.690064628731,164.688901078693,165.687737528655,166.686573978617,167.685410428579,
168.684246878541,169.683083328503,170.681919778464,171.680756228426,172.679592678388,
173.67842912835,174.677265578312,175.676102028274,176.674938478236,177.673774928198,
178.672611378159,179.671447828121,180.670284278083,181.669120728045,182.667957178007,
183.666793627969,184.665630077931,185.664466527893,186.663302977854),
 .UNSPECIFIED.);
#156=B_SPLINE_SURFACE_WITH_KNOTS('',3,3,((#120045,#120046,#120047,#120048,
#120049,#120050,#120051,#120052,#120053,#120054,#120055,#120056,#120057,
#120058,#120059,#120060,#120061,#120062,#120063,#120064,#120065,#120066,
#120067,#120068,#120069,#120070,#120071,#120072,#120073,#120074,#120075,
#120076,#120077,#120078,#120079,#120080,#120081,#120082,#120083,#120084,
#120085,#120086,#120087,#120088,#120089,#120090,#120091,#120092,#120093,
#120094,#120095,#120096,#120097,#120098,#120099,#120100,#120101,#120102,
#120103,#120104,#120105,#120106,#120107,#120108,#120109,#120110,#120111,
#120112,#120113,#120114,#120115,#120116,#120117,#120118,#120119,#120120,
#120121,#120122,#120123,#120124,#120125,#120126,#120127,#120128,#120129,
#120130,#120131,#120132,#120133,#120134,#120135,#120136,#120137,#120138,
#120139,#120140,#120141,#120142,#120143,#120144,#120145,#120146,#120147,
#120148,#120149,#120150,#120151,#120152,#120153,#120154,#120155,#120156,
#120157,#120158,#120159,#120160,#120161,#120162,#120163,#120164,#120165,
#120166,#120167,#120168,#120169,#120170,#120171,#120172,#120173,#120174,
#120175,#120176,#120177,#120178,#120179,#120180,#120181,#120182,#120183,
#120184,#120185,#120186,#120187,#120188,#120189,#120190,#120191,#120192,
#120193,#120194,#120195,#120196,#120197,#120198,#120199,#120200,#120201,
#120202,#120203,#120204,#120205,#120206,#120207,#120208,#120209,#120210,
#120211,#120212,#120213,#120214,#120215,#120216,#120217,#120218,#120219,
#120220,#120221,#120222),(#120223,#120224,#120225,#120226,#120227,#120228,
#120229,#120230,#120231,#120232,#120233,#120234,#120235,#120236,#120237,
#120238,#120239,#120240,#120241,#120242,#120243,#120244,#120245,#120246,
#120247,#120248,#120249,#120250,#120251,#120252,#120253,#120254,#120255,
#120256,#120257,#120258,#120259,#120260,#120261,#120262,#120263,#120264,
#120265,#120266,#120267,#120268,#120269,#120270,#120271,#120272,#120273,
#120274,#120275,#120276,#120277,#120278,#120279,#120280,#120281,#120282,
#120283,#120284,#120285,#120286,#120287,#120288,#120289,#120290,#120291,
#120292,#120293,#120294,#120295,#120296,#120297,#120298,#120299,#120300,
#120301,#120302,#120303,#120304,#120305,#120306,#120307,#120308,#120309,
#120310,#120311,#120312,#120313,#120314,#120315,#120316,#120317,#120318,
#120319,#120320,#120321,#120322,#120323,#120324,#120325,#120326,#120327,
#120328,#120329,#120330,#120331,#120332,#120333,#120334,#120335,#120336,
#120337,#120338,#120339,#120340,#120341,#120342,#120343,#120344,#120345,
#120346,#120347,#120348,#120349,#120350,#120351,#120352,#120353,#120354,
#120355,#120356,#120357,#120358,#120359,#120360,#120361,#120362,#120363,
#120364,#120365,#120366,#120367,#120368,#120369,#120370,#120371,#120372,
#120373,#120374,#120375,#120376,#120377,#120378,#120379,#120380,#120381,
#120382,#120383,#120384,#120385,#120386,#120387,#120388,#120389,#120390,
#120391,#120392,#120393,#120394,#120395,#120396,#120397,#120398,#120399,
#120400),(#120401,#120402,#120403,#120404,#120405,#120406,#120407,#120408,
#120409,#120410,#120411,#120412,#120413,#120414,#120415,#120416,#120417,
#120418,#120419,#120420,#120421,#120422,#120423,#120424,#120425,#120426,
#120427,#120428,#120429,#120430,#120431,#120432,#120433,#120434,#120435,
#120436,#120437,#120438,#120439,#120440,#120441,#120442,#120443,#120444,
#120445,#120446,#120447,#120448,#120449,#120450,#120451,#120452,#120453,
#120454,#120455,#120456,#120457,#120458,#120459,#120460,#120461,#120462,
#120463,#120464,#120465,#120466,#120467,#120468,#120469,#120470,#120471,
#120472,#120473,#120474,#120475,#120476,#120477,#120478,#120479,#120480,
#120481,#120482,#120483,#120484,#120485,#120486,#120487,#120488,#120489,
#120490,#120491,#120492,#120493,#120494,#120495,#120496,#120497,#120498,
#120499,#120500,#120501,#120502,#120503,#120504,#120505,#120506,#120507,
#120508,#120509,#120510,#120511,#120512,#120513,#120514,#120515,#120516,
#120517,#120518,#120519,#120520,#120521,#120522,#120523,#120524,#120525,
#120526,#120527,#120528,#120529,#120530,#120531,#120532,#120533,#120534,
#120535,#120536,#120537,#120538,#120539,#120540,#120541,#120542,#120543,
#120544,#120545,#120546,#120547,#120548,#120549,#120550,#120551,#120552,
#120553,#120554,#120555,#120556,#120557,#120558,#120559,#120560,#120561,
#120562,#120563,#120564,#120565,#120566,#120567,#120568,#120569,#120570,
#120571,#120572,#120573,#120574,#120575,#120576,#120577,#120578),(#120579,
#120580,#120581,#120582,#120583,#120584,#120585,#120586,#120587,#120588,
#120589,#120590,#120591,#120592,#120593,#120594,#120595,#120596,#120597,
#120598,#120599,#120600,#120601,#120602,#120603,#120604,#120605,#120606,
#120607,#120608,#120609,#120610,#120611,#120612,#120613,#120614,#120615,
#120616,#120617,#120618,#120619,#120620,#120621,#120622,#120623,#120624,
#120625,#120626,#120627,#120628,#120629,#120630,#120631,#120632,#120633,
#120634,#120635,#120636,#120637,#120638,#120639,#120640,#120641,#120642,
#120643,#120644,#120645,#120646,#120647,#120648,#120649,#120650,#120651,
#120652,#120653,#120654,#120655,#120656,#120657,#120658,#120659,#120660,
#120661,#120662,#120663,#120664,#120665,#120666,#120667,#120668,#120669,
#120670,#120671,#120672,#120673,#120674,#120675,#120676,#120677,#120678,
#120679,#120680,#120681,#120682,#120683,#120684,#120685,#120686,#120687,
#120688,#120689,#120690,#120691,#120692,#120693,#120694,#120695,#120696,
#120697,#120698,#120699,#120700,#120701,#120702,#120703,#120704,#120705,
#120706,#120707,#120708,#120709,#120710,#120711,#120712,#120713,#120714,
#120715,#120716,#120717,#120718,#120719,#120720,#120721,#120722,#120723,
#120724,#120725,#120726,#120727,#120728,#120729,#120730,#120731,#120732,
#120733,#120734,#120735,#120736,#120737,#120738,#120739,#120740,#120741,
#120742,#120743,#120744,#120745,#120746,#120747,#120748,#120749,#120750,
#120751,#120752,#120753,#120754,#120755,#120756)),.UNSPECIFIED.,.F.,.F.,
 .F.,(4,4),(4,1,1,1,1,1,1,1,1,1,1,1,1,1,1,1,1,1,1,1,1,1,1,1,1,1,1,1,1,1,
1,1,1,1,1,1,1,1,1,1,1,1,1,1,1,1,1,1,1,1,1,1,1,1,1,1,1,1,1,1,1,1,1,1,1,1,
1,1,1,1,1,1,1,1,1,1,1,1,1,1,1,1,1,1,1,1,1,1,1,1,1,1,1,1,1,1,1,1,1,1,1,1,
1,1,1,1,1,1,1,1,1,1,1,1,1,1,1,1,1,1,1,1,1,1,1,1,1,1,1,1,1,1,1,1,1,1,1,1,
1,1,1,1,1,1,1,1,1,1,1,1,1,1,1,1,1,1,1,1,1,1,1,1,1,1,1,1,1,1,1,1,1,1,1,1,
1,4),(-0.000378192696996877,0.0515928473073541),(14.3986268518925,15.3974633018543,
16.3962997518162,17.3951362017781,18.39397265174,19.3928091017018,20.3916455516637,
21.3904820016256,22.3893184515875,23.3881549015493,24.3869913515112,25.3858278014731,
26.3846642514349,27.3835007013968,28.3823371513587,29.3811736013206,30.3800100512824,
31.3788465012443,32.3776829512062,33.3765194011681,34.3753558511299,35.3741923010918,
36.3730287510537,37.3718652010156,38.3707016509774,39.3695381009393,40.3683745509012,
41.3672110008631,42.3660474508249,43.3648839007868,44.3637203507487,45.3625568007106,
46.3613932506724,47.3602297006343,48.3590661505962,49.3579026005581,50.3567390505199,
51.3555755004818,52.3544119504437,53.3532484004055,54.3520848503674,55.3509213003293,
56.3497577502912,57.348594200253,58.3474306502149,59.3462671001768,60.3451035501387,
61.3439400001005,62.3427764500624,63.3416129000243,64.3404493499862,65.339285799948,
66.3381222499099,67.3369586998718,68.3357951498337,69.3346315997955,70.3334680497574,
71.3323044997193,72.3311409496812,73.329977399643,74.3288138496049,75.3276502995668,
76.3264867495287,77.3253231994905,78.3241596494524,79.3229960994143,80.3218325493762,
81.320668999338,82.3195054492999,83.3183418992618,84.3171783492237,85.3160147991855,
86.3148512491474,87.3136876991093,88.3125241490712,89.311360599033,90.3101970489949,
91.3090334989568,92.3078699489186,93.3067063988805,94.3055428488424,95.3043792988043,
96.3032157487661,97.302052198728,98.3008886486899,99.2997250986518,100.298561548614,
101.297397998576,102.296234448537,103.295070898499,104.293907348461,105.292743798423,
106.291580248385,107.290416698347,108.289253148309,109.288089598271,110.286926048232,
111.285762498194,112.284598948156,113.283435398118,114.28227184808,115.281108298042,
116.279944748004,117.278781197966,118.277617647927,119.276454097889,120.275290547851,
121.274126997813,122.272963447775,123.271799897737,124.270636347699,125.26947279766,
126.268309247622,127.267145697584,128.265982147546,129.264818597508,130.26365504747,
131.262491497432,132.261327947394,133.260164397355,134.259000847317,135.257837297279,
136.256673747241,137.255510197203,138.254346647165,139.253183097127,140.252019547089,
141.25085599705,142.249692447012,143.248528896974,144.247365346936,145.246201796898,
146.24503824686,147.243874696822,148.242711146784,149.241547596745,150.240384046707,
151.239220496669,152.238056946631,153.236893396593,154.235729846555,155.234566296517,
156.233402746479,157.23223919644,158.231075646402,159.229912096364,160.228748546326,
161.227584996288,162.22642144625,163.225257896212,164.224094346174,165.222930796135,
166.221767246097,167.220603696059,168.219440146021,169.218276595983,170.217113045945,
171.215949495907,172.214785945869,173.21362239583,174.212458845792,175.211295295754,
176.210131745716,177.208968195678,178.20780464564,179.206641095602,180.205477545564,
181.204313995525,182.203150445487,183.201986895449,184.200823345411,185.199659795373,
186.198496245335,187.197332695297,188.196169145259,189.195445208677),
 .UNSPECIFIED.);
#157=B_SPLINE_SURFACE_WITH_KNOTS('',3,3,((#120845,#120846,#120847,#120848,
#120849,#120850,#120851,#120852,#120853,#120854,#120855,#120856,#120857,
#120858,#120859,#120860,#120861,#120862,#120863,#120864,#120865,#120866,
#120867,#120868,#120869,#120870,#120871,#120872,#120873,#120874,#120875,
#120876,#120877,#120878,#120879,#120880,#120881,#120882,#120883,#120884,
#120885,#120886,#120887,#120888,#120889,#120890,#120891,#120892,#120893,
#120894,#120895,#120896,#120897,#120898,#120899,#120900,#120901,#120902,
#120903,#120904,#120905,#120906,#120907,#120908,#120909,#120910,#120911,
#120912,#120913,#120914,#120915,#120916,#120917,#120918,#120919,#120920,
#120921,#120922,#120923,#120924,#120925,#120926,#120927,#120928,#120929,
#120930,#120931,#120932,#120933,#120934,#120935,#120936,#120937,#120938,
#120939,#120940,#120941,#120942,#120943,#120944,#120945,#120946,#120947,
#120948,#120949,#120950,#120951,#120952,#120953,#120954,#120955,#120956,
#120957,#120958,#120959,#120960,#120961,#120962,#120963,#120964,#120965,
#120966,#120967,#120968,#120969,#120970,#120971,#120972,#120973,#120974,
#120975,#120976,#120977,#120978,#120979,#120980,#120981,#120982,#120983,
#120984,#120985,#120986,#120987,#120988,#120989,#120990,#120991,#120992,
#120993,#120994,#120995,#120996,#120997,#120998,#120999,#121000,#121001,
#121002,#121003,#121004,#121005,#121006,#121007,#121008,#121009,#121010,
#121011,#121012,#121013,#121014,#121015,#121016,#121017,#121018,#121019,
#121020,#121021,#121022),(#121023,#121024,#121025,#121026,#121027,#121028,
#121029,#121030,#121031,#121032,#121033,#121034,#121035,#121036,#121037,
#121038,#121039,#121040,#121041,#121042,#121043,#121044,#121045,#121046,
#121047,#121048,#121049,#121050,#121051,#121052,#121053,#121054,#121055,
#121056,#121057,#121058,#121059,#121060,#121061,#121062,#121063,#121064,
#121065,#121066,#121067,#121068,#121069,#121070,#121071,#121072,#121073,
#121074,#121075,#121076,#121077,#121078,#121079,#121080,#121081,#121082,
#121083,#121084,#121085,#121086,#121087,#121088,#121089,#121090,#121091,
#121092,#121093,#121094,#121095,#121096,#121097,#121098,#121099,#121100,
#121101,#121102,#121103,#121104,#121105,#121106,#121107,#121108,#121109,
#121110,#121111,#121112,#121113,#121114,#121115,#121116,#121117,#121118,
#121119,#121120,#121121,#121122,#121123,#121124,#121125,#121126,#121127,
#121128,#121129,#121130,#121131,#121132,#121133,#121134,#121135,#121136,
#121137,#121138,#121139,#121140,#121141,#121142,#121143,#121144,#121145,
#121146,#121147,#121148,#121149,#121150,#121151,#121152,#121153,#121154,
#121155,#121156,#121157,#121158,#121159,#121160,#121161,#121162,#121163,
#121164,#121165,#121166,#121167,#121168,#121169,#121170,#121171,#121172,
#121173,#121174,#121175,#121176,#121177,#121178,#121179,#121180,#121181,
#121182,#121183,#121184,#121185,#121186,#121187,#121188,#121189,#121190,
#121191,#121192,#121193,#121194,#121195,#121196,#121197,#121198,#121199,
#121200),(#121201,#121202,#121203,#121204,#121205,#121206,#121207,#121208,
#121209,#121210,#121211,#121212,#121213,#121214,#121215,#121216,#121217,
#121218,#121219,#121220,#121221,#121222,#121223,#121224,#121225,#121226,
#121227,#121228,#121229,#121230,#121231,#121232,#121233,#121234,#121235,
#121236,#121237,#121238,#121239,#121240,#121241,#121242,#121243,#121244,
#121245,#121246,#121247,#121248,#121249,#121250,#121251,#121252,#121253,
#121254,#121255,#121256,#121257,#121258,#121259,#121260,#121261,#121262,
#121263,#121264,#121265,#121266,#121267,#121268,#121269,#121270,#121271,
#121272,#121273,#121274,#121275,#121276,#121277,#121278,#121279,#121280,
#121281,#121282,#121283,#121284,#121285,#121286,#121287,#121288,#121289,
#121290,#121291,#121292,#121293,#121294,#121295,#121296,#121297,#121298,
#121299,#121300,#121301,#121302,#121303,#121304,#121305,#121306,#121307,
#121308,#121309,#121310,#121311,#121312,#121313,#121314,#121315,#121316,
#121317,#121318,#121319,#121320,#121321,#121322,#121323,#121324,#121325,
#121326,#121327,#121328,#121329,#121330,#121331,#121332,#121333,#121334,
#121335,#121336,#121337,#121338,#121339,#121340,#121341,#121342,#121343,
#121344,#121345,#121346,#121347,#121348,#121349,#121350,#121351,#121352,
#121353,#121354,#121355,#121356,#121357,#121358,#121359,#121360,#121361,
#121362,#121363,#121364,#121365,#121366,#121367,#121368,#121369,#121370,
#121371,#121372,#121373,#121374,#121375,#121376,#121377,#121378),(#121379,
#121380,#121381,#121382,#121383,#121384,#121385,#121386,#121387,#121388,
#121389,#121390,#121391,#121392,#121393,#121394,#121395,#121396,#121397,
#121398,#121399,#121400,#121401,#121402,#121403,#121404,#121405,#121406,
#121407,#121408,#121409,#121410,#121411,#121412,#121413,#121414,#121415,
#121416,#121417,#121418,#121419,#121420,#121421,#121422,#121423,#121424,
#121425,#121426,#121427,#121428,#121429,#121430,#121431,#121432,#121433,
#121434,#121435,#121436,#121437,#121438,#121439,#121440,#121441,#121442,
#121443,#121444,#121445,#121446,#121447,#121448,#121449,#121450,#121451,
#121452,#121453,#121454,#121455,#121456,#121457,#121458,#121459,#121460,
#121461,#121462,#121463,#121464,#121465,#121466,#121467,#121468,#121469,
#121470,#121471,#121472,#121473,#121474,#121475,#121476,#121477,#121478,
#121479,#121480,#121481,#121482,#121483,#121484,#121485,#121486,#121487,
#121488,#121489,#121490,#121491,#121492,#121493,#121494,#121495,#121496,
#121497,#121498,#121499,#121500,#121501,#121502,#121503,#121504,#121505,
#121506,#121507,#121508,#121509,#121510,#121511,#121512,#121513,#121514,
#121515,#121516,#121517,#121518,#121519,#121520,#121521,#121522,#121523,
#121524,#121525,#121526,#121527,#121528,#121529,#121530,#121531,#121532,
#121533,#121534,#121535,#121536,#121537,#121538,#121539,#121540,#121541,
#121542,#121543,#121544,#121545,#121546,#121547,#121548,#121549,#121550,
#121551,#121552,#121553,#121554,#121555,#121556)),.UNSPECIFIED.,.F.,.F.,
 .F.,(4,4),(4,1,1,1,1,1,1,1,1,1,1,1,1,1,1,1,1,1,1,1,1,1,1,1,1,1,1,1,1,1,
1,1,1,1,1,1,1,1,1,1,1,1,1,1,1,1,1,1,1,1,1,1,1,1,1,1,1,1,1,1,1,1,1,1,1,1,
1,1,1,1,1,1,1,1,1,1,1,1,1,1,1,1,1,1,1,1,1,1,1,1,1,1,1,1,1,1,1,1,1,1,1,1,
1,1,1,1,1,1,1,1,1,1,1,1,1,1,1,1,1,1,1,1,1,1,1,1,1,1,1,1,1,1,1,1,1,1,1,1,
1,1,1,1,1,1,1,1,1,1,1,1,1,1,1,1,1,1,1,1,1,1,1,1,1,1,1,1,1,1,1,1,1,1,1,1,
1,4),(-0.000439572128271918,0.0515314616970906),(11.8664846623981,12.8657606844883,
13.8645971344502,14.8634335844121,15.8622700343739,16.8611064843358,17.8599429342977,
18.8587793842596,19.8576158342214,20.8564522841833,21.8552887341452,22.854125184107,
23.8529616340689,24.8517980840308,25.8506345339927,26.8494709839545,27.8483074339164,
28.8471438838783,29.8459803338402,30.844816783802,31.8436532337639,32.8424896837258,
33.8413261336877,34.8401625836495,35.8389990336114,36.8378354835733,37.8366719335352,
38.835508383497,39.8343448334589,40.8331812834208,41.8320177333827,42.8308541833445,
43.8296906333064,44.8285270832683,45.8273635332302,46.826199983192,47.8250364331539,
48.8238728831158,49.8227093330777,50.8215457830395,51.8203822330014,52.8192186829633,
53.8180551329252,54.816891582887,55.8157280328489,56.8145644828108,57.8134009327727,
58.8122373827345,59.8110738326964,60.8099102826583,61.8087467326202,62.807583182582,
63.8064196325439,64.8052560825058,65.8040925324676,66.8029289824295,67.8017654323914,
68.8006018823533,69.7994383323151,70.798274782277,71.7971112322389,72.7959476822008,
73.7947841321626,74.7936205821245,75.7924570320864,76.7912934820483,77.7901299320101,
78.788966381972,79.7878028319339,80.7866392818958,81.7854757318576,82.7843121818195,
83.7831486317814,84.7819850817433,85.7808215317051,86.779657981667,87.7784944316289,
88.7773308815908,89.7761673315526,90.7750037815145,91.7738402314764,92.7726766814383,
93.7715131314001,94.770349581362,95.7691860313239,96.7680224812858,97.7668589312476,
98.7656953812095,99.7645318311714,100.763368281133,101.762204731095,102.761041181057,
103.759877631019,104.758714080981,105.757550530943,106.756386980905,107.755223430866,
108.754059880828,109.75289633079,110.751732780752,111.750569230714,112.749405680676,
113.748242130638,114.747078580599,115.745915030561,116.744751480523,117.743587930485,
118.742424380447,119.741260830409,120.740097280371,121.738933730333,122.737770180294,
123.736606630256,124.735443080218,125.73427953018,126.733115980142,127.731952430104,
128.730788880066,129.729625330028,130.728461779989,131.727298229951,132.726134679913,
133.724971129875,134.723807579837,135.722644029799,136.721480479761,137.720316929723,
138.719153379684,139.717989829646,140.716826279608,141.71566272957,142.714499179532,
143.713335629494,144.712172079456,145.711008529418,146.709844979379,147.708681429341,
148.707517879303,149.706354329265,150.705190779227,151.704027229189,152.702863679151,
153.701700129113,154.700536579074,155.699373029036,156.698209478998,157.69704592896,
158.695882378922,159.694718828884,160.693555278846,161.692391728808,162.691228178769,
163.690064628731,164.688901078693,165.687737528655,166.686573978617,167.685410428579,
168.684246878541,169.683083328503,170.681919778464,171.680756228426,172.679592678388,
173.67842912835,174.677265578312,175.676102028274,176.674938478236,177.673774928198,
178.672611378159,179.671447828121,180.670284278083,181.669120728045,182.667957178007,
183.666793627969,184.665630077931,185.664466527893,186.663302977854),
 .UNSPECIFIED.);
#158=B_SPLINE_SURFACE_WITH_KNOTS('',3,3,((#121645,#121646,#121647,#121648,
#121649,#121650,#121651,#121652,#121653,#121654,#121655,#121656,#121657,
#121658,#121659,#121660,#121661,#121662,#121663,#121664,#121665,#121666,
#121667,#121668,#121669,#121670,#121671,#121672,#121673,#121674,#121675,
#121676,#121677,#121678,#121679,#121680,#121681,#121682,#121683,#121684,
#121685,#121686,#121687,#121688,#121689,#121690,#121691,#121692,#121693,
#121694,#121695,#121696,#121697,#121698,#121699,#121700,#121701,#121702,
#121703,#121704,#121705,#121706,#121707,#121708,#121709,#121710,#121711,
#121712,#121713,#121714,#121715,#121716,#121717,#121718,#121719,#121720,
#121721,#121722,#121723,#121724,#121725,#121726,#121727,#121728,#121729,
#121730,#121731,#121732,#121733,#121734,#121735,#121736,#121737,#121738,
#121739,#121740,#121741,#121742,#121743,#121744,#121745,#121746,#121747,
#121748,#121749,#121750,#121751,#121752,#121753,#121754,#121755,#121756,
#121757,#121758,#121759,#121760,#121761,#121762,#121763,#121764,#121765,
#121766,#121767,#121768,#121769,#121770,#121771,#121772,#121773,#121774,
#121775,#121776,#121777,#121778,#121779,#121780,#121781,#121782,#121783,
#121784,#121785,#121786,#121787,#121788,#121789,#121790,#121791,#121792,
#121793,#121794,#121795,#121796,#121797,#121798,#121799,#121800,#121801,
#121802,#121803,#121804,#121805,#121806,#121807,#121808,#121809,#121810,
#121811,#121812,#121813,#121814,#121815,#121816,#121817,#121818,#121819,
#121820,#121821,#121822),(#121823,#121824,#121825,#121826,#121827,#121828,
#121829,#121830,#121831,#121832,#121833,#121834,#121835,#121836,#121837,
#121838,#121839,#121840,#121841,#121842,#121843,#121844,#121845,#121846,
#121847,#121848,#121849,#121850,#121851,#121852,#121853,#121854,#121855,
#121856,#121857,#121858,#121859,#121860,#121861,#121862,#121863,#121864,
#121865,#121866,#121867,#121868,#121869,#121870,#121871,#121872,#121873,
#121874,#121875,#121876,#121877,#121878,#121879,#121880,#121881,#121882,
#121883,#121884,#121885,#121886,#121887,#121888,#121889,#121890,#121891,
#121892,#121893,#121894,#121895,#121896,#121897,#121898,#121899,#121900,
#121901,#121902,#121903,#121904,#121905,#121906,#121907,#121908,#121909,
#121910,#121911,#121912,#121913,#121914,#121915,#121916,#121917,#121918,
#121919,#121920,#121921,#121922,#121923,#121924,#121925,#121926,#121927,
#121928,#121929,#121930,#121931,#121932,#121933,#121934,#121935,#121936,
#121937,#121938,#121939,#121940,#121941,#121942,#121943,#121944,#121945,
#121946,#121947,#121948,#121949,#121950,#121951,#121952,#121953,#121954,
#121955,#121956,#121957,#121958,#121959,#121960,#121961,#121962,#121963,
#121964,#121965,#121966,#121967,#121968,#121969,#121970,#121971,#121972,
#121973,#121974,#121975,#121976,#121977,#121978,#121979,#121980,#121981,
#121982,#121983,#121984,#121985,#121986,#121987,#121988,#121989,#121990,
#121991,#121992,#121993,#121994,#121995,#121996,#121997,#121998,#121999,
#122000),(#122001,#122002,#122003,#122004,#122005,#122006,#122007,#122008,
#122009,#122010,#122011,#122012,#122013,#122014,#122015,#122016,#122017,
#122018,#122019,#122020,#122021,#122022,#122023,#122024,#122025,#122026,
#122027,#122028,#122029,#122030,#122031,#122032,#122033,#122034,#122035,
#122036,#122037,#122038,#122039,#122040,#122041,#122042,#122043,#122044,
#122045,#122046,#122047,#122048,#122049,#122050,#122051,#122052,#122053,
#122054,#122055,#122056,#122057,#122058,#122059,#122060,#122061,#122062,
#122063,#122064,#122065,#122066,#122067,#122068,#122069,#122070,#122071,
#122072,#122073,#122074,#122075,#122076,#122077,#122078,#122079,#122080,
#122081,#122082,#122083,#122084,#122085,#122086,#122087,#122088,#122089,
#122090,#122091,#122092,#122093,#122094,#122095,#122096,#122097,#122098,
#122099,#122100,#122101,#122102,#122103,#122104,#122105,#122106,#122107,
#122108,#122109,#122110,#122111,#122112,#122113,#122114,#122115,#122116,
#122117,#122118,#122119,#122120,#122121,#122122,#122123,#122124,#122125,
#122126,#122127,#122128,#122129,#122130,#122131,#122132,#122133,#122134,
#122135,#122136,#122137,#122138,#122139,#122140,#122141,#122142,#122143,
#122144,#122145,#122146,#122147,#122148,#122149,#122150,#122151,#122152,
#122153,#122154,#122155,#122156,#122157,#122158,#122159,#122160,#122161,
#122162,#122163,#122164,#122165,#122166,#122167,#122168,#122169,#122170,
#122171,#122172,#122173,#122174,#122175,#122176,#122177,#122178),(#122179,
#122180,#122181,#122182,#122183,#122184,#122185,#122186,#122187,#122188,
#122189,#122190,#122191,#122192,#122193,#122194,#122195,#122196,#122197,
#122198,#122199,#122200,#122201,#122202,#122203,#122204,#122205,#122206,
#122207,#122208,#122209,#122210,#122211,#122212,#122213,#122214,#122215,
#122216,#122217,#122218,#122219,#122220,#122221,#122222,#122223,#122224,
#122225,#122226,#122227,#122228,#122229,#122230,#122231,#122232,#122233,
#122234,#122235,#122236,#122237,#122238,#122239,#122240,#122241,#122242,
#122243,#122244,#122245,#122246,#122247,#122248,#122249,#122250,#122251,
#122252,#122253,#122254,#122255,#122256,#122257,#122258,#122259,#122260,
#122261,#122262,#122263,#122264,#122265,#122266,#122267,#122268,#122269,
#122270,#122271,#122272,#122273,#122274,#122275,#122276,#122277,#122278,
#122279,#122280,#122281,#122282,#122283,#122284,#122285,#122286,#122287,
#122288,#122289,#122290,#122291,#122292,#122293,#122294,#122295,#122296,
#122297,#122298,#122299,#122300,#122301,#122302,#122303,#122304,#122305,
#122306,#122307,#122308,#122309,#122310,#122311,#122312,#122313,#122314,
#122315,#122316,#122317,#122318,#122319,#122320,#122321,#122322,#122323,
#122324,#122325,#122326,#122327,#122328,#122329,#122330,#122331,#122332,
#122333,#122334,#122335,#122336,#122337,#122338,#122339,#122340,#122341,
#122342,#122343,#122344,#122345,#122346,#122347,#122348,#122349,#122350,
#122351,#122352,#122353,#122354,#122355,#122356)),.UNSPECIFIED.,.F.,.F.,
 .F.,(4,4),(4,1,1,1,1,1,1,1,1,1,1,1,1,1,1,1,1,1,1,1,1,1,1,1,1,1,1,1,1,1,
1,1,1,1,1,1,1,1,1,1,1,1,1,1,1,1,1,1,1,1,1,1,1,1,1,1,1,1,1,1,1,1,1,1,1,1,
1,1,1,1,1,1,1,1,1,1,1,1,1,1,1,1,1,1,1,1,1,1,1,1,1,1,1,1,1,1,1,1,1,1,1,1,
1,1,1,1,1,1,1,1,1,1,1,1,1,1,1,1,1,1,1,1,1,1,1,1,1,1,1,1,1,1,1,1,1,1,1,1,
1,1,1,1,1,1,1,1,1,1,1,1,1,1,1,1,1,1,1,1,1,1,1,1,1,1,1,1,1,1,1,1,1,1,1,1,
1,4),(-0.000378196170333863,0.0515928432182127),(14.3986268518925,15.3974633018543,
16.3962997518162,17.3951362017781,18.39397265174,19.3928091017018,20.3916455516637,
21.3904820016256,22.3893184515875,23.3881549015493,24.3869913515112,25.3858278014731,
26.384664251435,27.3835007013968,28.3823371513587,29.3811736013206,30.3800100512825,
31.3788465012443,32.3776829512062,33.3765194011681,34.37535585113,35.3741923010918,
36.3730287510537,37.3718652010156,38.3707016509774,39.3695381009393,40.3683745509012,
41.3672110008631,42.3660474508249,43.3648839007868,44.3637203507487,45.3625568007106,
46.3613932506724,47.3602297006343,48.3590661505962,49.3579026005581,50.3567390505199,
51.3555755004818,52.3544119504437,53.3532484004056,54.3520848503674,55.3509213003293,
56.3497577502912,57.3485942002531,58.3474306502149,59.3462671001768,60.3451035501387,
61.3439400001006,62.3427764500624,63.3416129000243,64.3404493499862,65.3392857999481,
66.3381222499099,67.3369586998718,68.3357951498337,69.3346315997956,70.3334680497574,
71.3323044997193,72.3311409496812,73.3299773996431,74.3288138496049,75.3276502995668,
76.3264867495287,77.3253231994906,78.3241596494524,79.3229960994143,80.3218325493762,
81.3206689993381,82.3195054492999,83.3183418992618,84.3171783492237,85.3160147991856,
86.3148512491474,87.3136876991093,88.3125241490712,89.3113605990331,90.3101970489949,
91.3090334989568,92.3078699489187,93.3067063988806,94.3055428488424,95.3043792988043,
96.3032157487662,97.302052198728,98.3008886486899,99.2997250986518,100.298561548614,
101.297397998576,102.296234448537,103.295070898499,104.293907348461,105.292743798423,
106.291580248385,107.290416698347,108.289253148309,109.288089598271,110.286926048232,
111.285762498194,112.284598948156,113.283435398118,114.28227184808,115.281108298042,
116.279944748004,117.278781197966,118.277617647927,119.276454097889,120.275290547851,
121.274126997813,122.272963447775,123.271799897737,124.270636347699,125.269472797661,
126.268309247622,127.267145697584,128.265982147546,129.264818597508,130.26365504747,
131.262491497432,132.261327947394,133.260164397356,134.259000847317,135.257837297279,
136.256673747241,137.255510197203,138.254346647165,139.253183097127,140.252019547089,
141.250855997051,142.249692447012,143.248528896974,144.247365346936,145.246201796898,
146.24503824686,147.243874696822,148.242711146784,149.241547596746,150.240384046707,
151.239220496669,152.238056946631,153.236893396593,154.235729846555,155.234566296517,
156.233402746479,157.232239196441,158.231075646402,159.229912096364,160.228748546326,
161.227584996288,162.22642144625,163.225257896212,164.224094346174,165.222930796136,
166.221767246097,167.220603696059,168.219440146021,169.218276595983,170.217113045945,
171.215949495907,172.214785945869,173.21362239583,174.212458845792,175.211295295754,
176.210131745716,177.208968195678,178.20780464564,179.206641095602,180.205477545564,
181.204313995525,182.203150445487,183.201986895449,184.200823345411,185.199659795373,
186.198496245335,187.197332695297,188.196169145259,189.195445204588),
 .UNSPECIFIED.);
#159=B_SPLINE_SURFACE_WITH_KNOTS('',3,3,((#122445,#122446,#122447,#122448,
#122449,#122450,#122451,#122452,#122453,#122454,#122455,#122456,#122457,
#122458,#122459,#122460,#122461,#122462,#122463,#122464,#122465,#122466,
#122467,#122468,#122469,#122470,#122471,#122472,#122473,#122474,#122475,
#122476,#122477,#122478,#122479,#122480,#122481,#122482,#122483,#122484,
#122485,#122486,#122487,#122488,#122489,#122490,#122491,#122492,#122493,
#122494,#122495,#122496,#122497,#122498,#122499,#122500,#122501,#122502,
#122503,#122504,#122505,#122506,#122507,#122508,#122509,#122510,#122511,
#122512,#122513,#122514,#122515,#122516,#122517,#122518,#122519,#122520,
#122521,#122522,#122523,#122524,#122525,#122526,#122527,#122528,#122529,
#122530,#122531,#122532,#122533,#122534,#122535,#122536,#122537,#122538,
#122539,#122540,#122541,#122542,#122543,#122544,#122545,#122546,#122547,
#122548,#122549,#122550,#122551,#122552,#122553,#122554,#122555,#122556,
#122557,#122558,#122559,#122560,#122561,#122562,#122563,#122564,#122565,
#122566,#122567,#122568,#122569,#122570,#122571,#122572,#122573,#122574,
#122575,#122576,#122577,#122578,#122579,#122580,#122581,#122582,#122583,
#122584,#122585,#122586,#122587,#122588,#122589,#122590,#122591,#122592,
#122593,#122594,#122595,#122596,#122597,#122598,#122599,#122600,#122601,
#122602,#122603,#122604,#122605,#122606,#122607,#122608,#122609,#122610,
#122611,#122612,#122613,#122614,#122615,#122616,#122617,#122618,#122619,
#122620,#122621,#122622),(#122623,#122624,#122625,#122626,#122627,#122628,
#122629,#122630,#122631,#122632,#122633,#122634,#122635,#122636,#122637,
#122638,#122639,#122640,#122641,#122642,#122643,#122644,#122645,#122646,
#122647,#122648,#122649,#122650,#122651,#122652,#122653,#122654,#122655,
#122656,#122657,#122658,#122659,#122660,#122661,#122662,#122663,#122664,
#122665,#122666,#122667,#122668,#122669,#122670,#122671,#122672,#122673,
#122674,#122675,#122676,#122677,#122678,#122679,#122680,#122681,#122682,
#122683,#122684,#122685,#122686,#122687,#122688,#122689,#122690,#122691,
#122692,#122693,#122694,#122695,#122696,#122697,#122698,#122699,#122700,
#122701,#122702,#122703,#122704,#122705,#122706,#122707,#122708,#122709,
#122710,#122711,#122712,#122713,#122714,#122715,#122716,#122717,#122718,
#122719,#122720,#122721,#122722,#122723,#122724,#122725,#122726,#122727,
#122728,#122729,#122730,#122731,#122732,#122733,#122734,#122735,#122736,
#122737,#122738,#122739,#122740,#122741,#122742,#122743,#122744,#122745,
#122746,#122747,#122748,#122749,#122750,#122751,#122752,#122753,#122754,
#122755,#122756,#122757,#122758,#122759,#122760,#122761,#122762,#122763,
#122764,#122765,#122766,#122767,#122768,#122769,#122770,#122771,#122772,
#122773,#122774,#122775,#122776,#122777,#122778,#122779,#122780,#122781,
#122782,#122783,#122784,#122785,#122786,#122787,#122788,#122789,#122790,
#122791,#122792,#122793,#122794,#122795,#122796,#122797,#122798,#122799,
#122800),(#122801,#122802,#122803,#122804,#122805,#122806,#122807,#122808,
#122809,#122810,#122811,#122812,#122813,#122814,#122815,#122816,#122817,
#122818,#122819,#122820,#122821,#122822,#122823,#122824,#122825,#122826,
#122827,#122828,#122829,#122830,#122831,#122832,#122833,#122834,#122835,
#122836,#122837,#122838,#122839,#122840,#122841,#122842,#122843,#122844,
#122845,#122846,#122847,#122848,#122849,#122850,#122851,#122852,#122853,
#122854,#122855,#122856,#122857,#122858,#122859,#122860,#122861,#122862,
#122863,#122864,#122865,#122866,#122867,#122868,#122869,#122870,#122871,
#122872,#122873,#122874,#122875,#122876,#122877,#122878,#122879,#122880,
#122881,#122882,#122883,#122884,#122885,#122886,#122887,#122888,#122889,
#122890,#122891,#122892,#122893,#122894,#122895,#122896,#122897,#122898,
#122899,#122900,#122901,#122902,#122903,#122904,#122905,#122906,#122907,
#122908,#122909,#122910,#122911,#122912,#122913,#122914,#122915,#122916,
#122917,#122918,#122919,#122920,#122921,#122922,#122923,#122924,#122925,
#122926,#122927,#122928,#122929,#122930,#122931,#122932,#122933,#122934,
#122935,#122936,#122937,#122938,#122939,#122940,#122941,#122942,#122943,
#122944,#122945,#122946,#122947,#122948,#122949,#122950,#122951,#122952,
#122953,#122954,#122955,#122956,#122957,#122958,#122959,#122960,#122961,
#122962,#122963,#122964,#122965,#122966,#122967,#122968,#122969,#122970,
#122971,#122972,#122973,#122974,#122975,#122976,#122977,#122978),(#122979,
#122980,#122981,#122982,#122983,#122984,#122985,#122986,#122987,#122988,
#122989,#122990,#122991,#122992,#122993,#122994,#122995,#122996,#122997,
#122998,#122999,#123000,#123001,#123002,#123003,#123004,#123005,#123006,
#123007,#123008,#123009,#123010,#123011,#123012,#123013,#123014,#123015,
#123016,#123017,#123018,#123019,#123020,#123021,#123022,#123023,#123024,
#123025,#123026,#123027,#123028,#123029,#123030,#123031,#123032,#123033,
#123034,#123035,#123036,#123037,#123038,#123039,#123040,#123041,#123042,
#123043,#123044,#123045,#123046,#123047,#123048,#123049,#123050,#123051,
#123052,#123053,#123054,#123055,#123056,#123057,#123058,#123059,#123060,
#123061,#123062,#123063,#123064,#123065,#123066,#123067,#123068,#123069,
#123070,#123071,#123072,#123073,#123074,#123075,#123076,#123077,#123078,
#123079,#123080,#123081,#123082,#123083,#123084,#123085,#123086,#123087,
#123088,#123089,#123090,#123091,#123092,#123093,#123094,#123095,#123096,
#123097,#123098,#123099,#123100,#123101,#123102,#123103,#123104,#123105,
#123106,#123107,#123108,#123109,#123110,#123111,#123112,#123113,#123114,
#123115,#123116,#123117,#123118,#123119,#123120,#123121,#123122,#123123,
#123124,#123125,#123126,#123127,#123128,#123129,#123130,#123131,#123132,
#123133,#123134,#123135,#123136,#123137,#123138,#123139,#123140,#123141,
#123142,#123143,#123144,#123145,#123146,#123147,#123148,#123149,#123150,
#123151,#123152,#123153,#123154,#123155,#123156)),.UNSPECIFIED.,.F.,.F.,
 .F.,(4,4),(4,1,1,1,1,1,1,1,1,1,1,1,1,1,1,1,1,1,1,1,1,1,1,1,1,1,1,1,1,1,
1,1,1,1,1,1,1,1,1,1,1,1,1,1,1,1,1,1,1,1,1,1,1,1,1,1,1,1,1,1,1,1,1,1,1,1,
1,1,1,1,1,1,1,1,1,1,1,1,1,1,1,1,1,1,1,1,1,1,1,1,1,1,1,1,1,1,1,1,1,1,1,1,
1,1,1,1,1,1,1,1,1,1,1,1,1,1,1,1,1,1,1,1,1,1,1,1,1,1,1,1,1,1,1,1,1,1,1,1,
1,1,1,1,1,1,1,1,1,1,1,1,1,1,1,1,1,1,1,1,1,1,1,1,1,1,1,1,1,1,1,1,1,1,1,1,
1,4),(-0.000439583499978536,0.051531452015598),(11.8664846510264,12.8657606844883,
13.8645971344502,14.8634335844121,15.8622700343739,16.8611064843358,17.8599429342977,
18.8587793842596,19.8576158342214,20.8564522841833,21.8552887341452,22.854125184107,
23.8529616340689,24.8517980840308,25.8506345339927,26.8494709839545,27.8483074339164,
28.8471438838783,29.8459803338402,30.844816783802,31.8436532337639,32.8424896837258,
33.8413261336877,34.8401625836495,35.8389990336114,36.8378354835733,37.8366719335352,
38.835508383497,39.8343448334589,40.8331812834208,41.8320177333827,42.8308541833445,
43.8296906333064,44.8285270832683,45.8273635332302,46.826199983192,47.8250364331539,
48.8238728831158,49.8227093330777,50.8215457830395,51.8203822330014,52.8192186829633,
53.8180551329252,54.816891582887,55.8157280328489,56.8145644828108,57.8134009327727,
58.8122373827345,59.8110738326964,60.8099102826583,61.8087467326202,62.807583182582,
63.8064196325439,64.8052560825058,65.8040925324676,66.8029289824295,67.8017654323914,
68.8006018823533,69.7994383323151,70.798274782277,71.7971112322389,72.7959476822008,
73.7947841321626,74.7936205821245,75.7924570320864,76.7912934820483,77.7901299320101,
78.788966381972,79.7878028319339,80.7866392818958,81.7854757318576,82.7843121818195,
83.7831486317814,84.7819850817433,85.7808215317051,86.779657981667,87.7784944316289,
88.7773308815908,89.7761673315526,90.7750037815145,91.7738402314764,92.7726766814383,
93.7715131314001,94.770349581362,95.7691860313239,96.7680224812858,97.7668589312476,
98.7656953812095,99.7645318311714,100.763368281133,101.762204731095,102.761041181057,
103.759877631019,104.758714080981,105.757550530943,106.756386980905,107.755223430866,
108.754059880828,109.75289633079,110.751732780752,111.750569230714,112.749405680676,
113.748242130638,114.747078580599,115.745915030561,116.744751480523,117.743587930485,
118.742424380447,119.741260830409,120.740097280371,121.738933730333,122.737770180294,
123.736606630256,124.735443080218,125.73427953018,126.733115980142,127.731952430104,
128.730788880066,129.729625330028,130.728461779989,131.727298229951,132.726134679913,
133.724971129875,134.723807579837,135.722644029799,136.721480479761,137.720316929723,
138.719153379684,139.717989829646,140.716826279608,141.71566272957,142.714499179532,
143.713335629494,144.712172079456,145.711008529418,146.709844979379,147.708681429341,
148.707517879303,149.706354329265,150.705190779227,151.704027229189,152.702863679151,
153.701700129113,154.700536579074,155.699373029036,156.698209478998,157.69704592896,
158.695882378922,159.694718828884,160.693555278846,161.692391728808,162.691228178769,
163.690064628731,164.688901078693,165.687737528655,166.686573978617,167.685410428579,
168.684246878541,169.683083328503,170.681919778464,171.680756228426,172.679592678388,
173.67842912835,174.677265578312,175.676102028274,176.674938478236,177.673774928198,
178.672611378159,179.671447828121,180.670284278083,181.669120728045,182.667957178007,
183.666793627969,184.665630077931,185.664466527893,186.663302977854),
 .UNSPECIFIED.);
#160=B_SPLINE_SURFACE_WITH_KNOTS('',3,3,((#123242,#123243,#123244,#123245,
#123246,#123247,#123248,#123249,#123250,#123251,#123252,#123253,#123254,
#123255,#123256,#123257,#123258,#123259,#123260,#123261,#123262,#123263,
#123264,#123265,#123266,#123267,#123268,#123269,#123270,#123271,#123272,
#123273,#123274,#123275,#123276,#123277,#123278,#123279,#123280,#123281,
#123282,#123283,#123284,#123285,#123286,#123287,#123288,#123289,#123290,
#123291,#123292,#123293,#123294,#123295,#123296,#123297,#123298,#123299,
#123300,#123301,#123302,#123303,#123304,#123305,#123306,#123307,#123308,
#123309,#123310,#123311,#123312,#123313,#123314,#123315,#123316,#123317,
#123318,#123319,#123320,#123321,#123322,#123323,#123324,#123325,#123326,
#123327,#123328,#123329,#123330,#123331,#123332,#123333,#123334,#123335,
#123336,#123337,#123338,#123339,#123340,#123341,#123342,#123343,#123344,
#123345,#123346,#123347,#123348,#123349,#123350,#123351,#123352,#123353,
#123354,#123355,#123356,#123357,#123358,#123359,#123360,#123361,#123362,
#123363,#123364,#123365,#123366,#123367,#123368,#123369,#123370,#123371,
#123372,#123373,#123374,#123375,#123376,#123377,#123378,#123379,#123380,
#123381,#123382,#123383,#123384,#123385,#123386,#123387,#123388,#123389,
#123390,#123391,#123392,#123393,#123394,#123395,#123396,#123397,#123398,
#123399,#123400,#123401,#123402,#123403,#123404,#123405,#123406,#123407,
#123408,#123409,#123410,#123411,#123412,#123413,#123414,#123415,#123416,
#123417,#123418,#123419),(#123420,#123421,#123422,#123423,#123424,#123425,
#123426,#123427,#123428,#123429,#123430,#123431,#123432,#123433,#123434,
#123435,#123436,#123437,#123438,#123439,#123440,#123441,#123442,#123443,
#123444,#123445,#123446,#123447,#123448,#123449,#123450,#123451,#123452,
#123453,#123454,#123455,#123456,#123457,#123458,#123459,#123460,#123461,
#123462,#123463,#123464,#123465,#123466,#123467,#123468,#123469,#123470,
#123471,#123472,#123473,#123474,#123475,#123476,#123477,#123478,#123479,
#123480,#123481,#123482,#123483,#123484,#123485,#123486,#123487,#123488,
#123489,#123490,#123491,#123492,#123493,#123494,#123495,#123496,#123497,
#123498,#123499,#123500,#123501,#123502,#123503,#123504,#123505,#123506,
#123507,#123508,#123509,#123510,#123511,#123512,#123513,#123514,#123515,
#123516,#123517,#123518,#123519,#123520,#123521,#123522,#123523,#123524,
#123525,#123526,#123527,#123528,#123529,#123530,#123531,#123532,#123533,
#123534,#123535,#123536,#123537,#123538,#123539,#123540,#123541,#123542,
#123543,#123544,#123545,#123546,#123547,#123548,#123549,#123550,#123551,
#123552,#123553,#123554,#123555,#123556,#123557,#123558,#123559,#123560,
#123561,#123562,#123563,#123564,#123565,#123566,#123567,#123568,#123569,
#123570,#123571,#123572,#123573,#123574,#123575,#123576,#123577,#123578,
#123579,#123580,#123581,#123582,#123583,#123584,#123585,#123586,#123587,
#123588,#123589,#123590,#123591,#123592,#123593,#123594,#123595,#123596,
#123597),(#123598,#123599,#123600,#123601,#123602,#123603,#123604,#123605,
#123606,#123607,#123608,#123609,#123610,#123611,#123612,#123613,#123614,
#123615,#123616,#123617,#123618,#123619,#123620,#123621,#123622,#123623,
#123624,#123625,#123626,#123627,#123628,#123629,#123630,#123631,#123632,
#123633,#123634,#123635,#123636,#123637,#123638,#123639,#123640,#123641,
#123642,#123643,#123644,#123645,#123646,#123647,#123648,#123649,#123650,
#123651,#123652,#123653,#123654,#123655,#123656,#123657,#123658,#123659,
#123660,#123661,#123662,#123663,#123664,#123665,#123666,#123667,#123668,
#123669,#123670,#123671,#123672,#123673,#123674,#123675,#123676,#123677,
#123678,#123679,#123680,#123681,#123682,#123683,#123684,#123685,#123686,
#123687,#123688,#123689,#123690,#123691,#123692,#123693,#123694,#123695,
#123696,#123697,#123698,#123699,#123700,#123701,#123702,#123703,#123704,
#123705,#123706,#123707,#123708,#123709,#123710,#123711,#123712,#123713,
#123714,#123715,#123716,#123717,#123718,#123719,#123720,#123721,#123722,
#123723,#123724,#123725,#123726,#123727,#123728,#123729,#123730,#123731,
#123732,#123733,#123734,#123735,#123736,#123737,#123738,#123739,#123740,
#123741,#123742,#123743,#123744,#123745,#123746,#123747,#123748,#123749,
#123750,#123751,#123752,#123753,#123754,#123755,#123756,#123757,#123758,
#123759,#123760,#123761,#123762,#123763,#123764,#123765,#123766,#123767,
#123768,#123769,#123770,#123771,#123772,#123773,#123774,#123775),(#123776,
#123777,#123778,#123779,#123780,#123781,#123782,#123783,#123784,#123785,
#123786,#123787,#123788,#123789,#123790,#123791,#123792,#123793,#123794,
#123795,#123796,#123797,#123798,#123799,#123800,#123801,#123802,#123803,
#123804,#123805,#123806,#123807,#123808,#123809,#123810,#123811,#123812,
#123813,#123814,#123815,#123816,#123817,#123818,#123819,#123820,#123821,
#123822,#123823,#123824,#123825,#123826,#123827,#123828,#123829,#123830,
#123831,#123832,#123833,#123834,#123835,#123836,#123837,#123838,#123839,
#123840,#123841,#123842,#123843,#123844,#123845,#123846,#123847,#123848,
#123849,#123850,#123851,#123852,#123853,#123854,#123855,#123856,#123857,
#123858,#123859,#123860,#123861,#123862,#123863,#123864,#123865,#123866,
#123867,#123868,#123869,#123870,#123871,#123872,#123873,#123874,#123875,
#123876,#123877,#123878,#123879,#123880,#123881,#123882,#123883,#123884,
#123885,#123886,#123887,#123888,#123889,#123890,#123891,#123892,#123893,
#123894,#123895,#123896,#123897,#123898,#123899,#123900,#123901,#123902,
#123903,#123904,#123905,#123906,#123907,#123908,#123909,#123910,#123911,
#123912,#123913,#123914,#123915,#123916,#123917,#123918,#123919,#123920,
#123921,#123922,#123923,#123924,#123925,#123926,#123927,#123928,#123929,
#123930,#123931,#123932,#123933,#123934,#123935,#123936,#123937,#123938,
#123939,#123940,#123941,#123942,#123943,#123944,#123945,#123946,#123947,
#123948,#123949,#123950,#123951,#123952,#123953)),.UNSPECIFIED.,.F.,.F.,
 .F.,(4,4),(4,1,1,1,1,1,1,1,1,1,1,1,1,1,1,1,1,1,1,1,1,1,1,1,1,1,1,1,1,1,
1,1,1,1,1,1,1,1,1,1,1,1,1,1,1,1,1,1,1,1,1,1,1,1,1,1,1,1,1,1,1,1,1,1,1,1,
1,1,1,1,1,1,1,1,1,1,1,1,1,1,1,1,1,1,1,1,1,1,1,1,1,1,1,1,1,1,1,1,1,1,1,1,
1,1,1,1,1,1,1,1,1,1,1,1,1,1,1,1,1,1,1,1,1,1,1,1,1,1,1,1,1,1,1,1,1,1,1,1,
1,1,1,1,1,1,1,1,1,1,1,1,1,1,1,1,1,1,1,1,1,1,1,1,1,1,1,1,1,1,1,1,1,1,1,1,
1,4),(-0.000378221444736312,0.0515928134973294),(14.3986268518925,15.3974633018543,
16.3962997518162,17.3951362017781,18.39397265174,19.3928091017018,20.3916455516637,
21.3904820016256,22.3893184515875,23.3881549015493,24.3869913515112,25.3858278014731,
26.384664251435,27.3835007013968,28.3823371513587,29.3811736013206,30.3800100512825,
31.3788465012443,32.3776829512062,33.3765194011681,34.37535585113,35.3741923010918,
36.3730287510537,37.3718652010156,38.3707016509774,39.3695381009393,40.3683745509012,
41.3672110008631,42.3660474508249,43.3648839007868,44.3637203507487,45.3625568007106,
46.3613932506724,47.3602297006343,48.3590661505962,49.3579026005581,50.3567390505199,
51.3555755004818,52.3544119504437,53.3532484004056,54.3520848503674,55.3509213003293,
56.3497577502912,57.3485942002531,58.3474306502149,59.3462671001768,60.3451035501387,
61.3439400001006,62.3427764500624,63.3416129000243,64.3404493499862,65.3392857999481,
66.3381222499099,67.3369586998718,68.3357951498337,69.3346315997956,70.3334680497574,
71.3323044997193,72.3311409496812,73.3299773996431,74.3288138496049,75.3276502995668,
76.3264867495287,77.3253231994906,78.3241596494524,79.3229960994143,80.3218325493762,
81.3206689993381,82.3195054492999,83.3183418992618,84.3171783492237,85.3160147991856,
86.3148512491474,87.3136876991093,88.3125241490712,89.3113605990331,90.3101970489949,
91.3090334989568,92.3078699489187,93.3067063988806,94.3055428488424,95.3043792988043,
96.3032157487662,97.302052198728,98.3008886486899,99.2997250986518,100.298561548614,
101.297397998576,102.296234448537,103.295070898499,104.293907348461,105.292743798423,
106.291580248385,107.290416698347,108.289253148309,109.288089598271,110.286926048232,
111.285762498194,112.284598948156,113.283435398118,114.28227184808,115.281108298042,
116.279944748004,117.278781197966,118.277617647927,119.276454097889,120.275290547851,
121.274126997813,122.272963447775,123.271799897737,124.270636347699,125.269472797661,
126.268309247622,127.267145697584,128.265982147546,129.264818597508,130.26365504747,
131.262491497432,132.261327947394,133.260164397356,134.259000847317,135.257837297279,
136.256673747241,137.255510197203,138.254346647165,139.253183097127,140.252019547089,
141.250855997051,142.249692447012,143.248528896974,144.247365346936,145.246201796898,
146.24503824686,147.243874696822,148.242711146784,149.241547596746,150.240384046707,
151.239220496669,152.238056946631,153.236893396593,154.235729846555,155.234566296517,
156.233402746479,157.232239196441,158.231075646402,159.229912096364,160.228748546326,
161.227584996288,162.22642144625,163.225257896212,164.224094346174,165.222930796136,
166.221767246097,167.220603696059,168.219440146021,169.218276595983,170.217113045945,
171.215949495907,172.214785945869,173.21362239583,174.212458845792,175.211295295754,
176.210131745716,177.208968195678,178.20780464564,179.206641095602,180.205477545564,
181.204313995525,182.203150445487,183.201986895449,184.200823345411,185.199659795373,
186.198496245335,187.197332695297,188.196169145259,189.195445174867),
 .UNSPECIFIED.);
#173=FACE_BOUND('',#4590,.T.);
#174=FACE_BOUND('',#4591,.T.);
#175=FACE_BOUND('',#4592,.T.);
#176=FACE_BOUND('',#4593,.T.);
#177=FACE_BOUND('',#4594,.T.);
#178=FACE_BOUND('',#4595,.T.);
#179=FACE_BOUND('',#4596,.T.);
#180=FACE_BOUND('',#4597,.T.);
#181=FACE_BOUND('',#4598,.T.);
#182=FACE_BOUND('',#4620,.T.);
#183=FACE_BOUND('',#4627,.T.);
#184=FACE_BOUND('',#4628,.T.);
#185=FACE_BOUND('',#4629,.T.);
#186=FACE_BOUND('',#4639,.T.);
#187=FACE_BOUND('',#4653,.T.);
#188=FACE_BOUND('',#4654,.T.);
#189=FACE_BOUND('',#4655,.T.);
#190=FACE_BOUND('',#4665,.T.);
#191=FACE_BOUND('',#4675,.T.);
#192=FACE_BOUND('',#4679,.T.);
#193=FACE_BOUND('',#4680,.T.);
#194=FACE_BOUND('',#4703,.T.);
#195=FACE_BOUND('',#4704,.T.);
#196=FACE_BOUND('',#4715,.T.);
#197=FACE_BOUND('',#4716,.T.);
#198=FACE_BOUND('',#4717,.T.);
#199=FACE_BOUND('',#4718,.T.);
#247=B_SPLINE_CURVE_WITH_KNOTS('',3,(#36300,#36301,#36302,#36303,#36304,
#36305),.UNSPECIFIED.,.F.,.F.,(4,1,1,4),(36.782513561854,37.1950127479992,
37.6823602457602,38.1697077435212),.UNSPECIFIED.);
#248=B_SPLINE_CURVE_WITH_KNOTS('',3,(#36308,#36309,#36310,#36311,#36312,
#36313,#36314,#36315,#36316,#36317,#36318,#36319,#36320,#36321,#36322,#36323,
#36324,#36325,#36326,#36327,#36328,#36329,#36330,#36331,#36332,#36333,#36334,
#36335,#36336,#36337,#36338,#36339,#36340,#36341,#36342,#36343,#36344,#36345,
#36346,#36347,#36348,#36349,#36350,#36351,#36352,#36353,#36354,#36355,#36356,
#36357,#36358,#36359,#36360,#36361,#36362,#36363,#36364,#36365,#36366,#36367,
#36368,#36369,#36370,#36371,#36372,#36373,#36374,#36375,#36376,#36377,#36378,
#36379,#36380),.UNSPECIFIED.,.F.,.F.,(4,3,3,3,3,3,3,3,3,3,3,3,3,3,3,3,3,
3,3,3,3,3,3,3,4),(36.7824851161968,36.8175942235541,36.9047259080441,36.9918410494598,
37.0789592472834,37.166072719263,37.2532055288754,37.3049417213151,37.3920685377782,
37.4791788064371,37.5662921716237,37.6534008452347,37.7405289511405,37.7922892190762,
37.8794201571563,37.966534535352,38.0536519523545,38.1407646354665,38.2278966508317,
38.2796367168372,38.3664398614179,38.4532350920939,38.5400193187296,38.6268191082651,
38.6945925143091),.UNSPECIFIED.);
#249=B_SPLINE_CURVE_WITH_KNOTS('',3,(#36386,#36387,#36388,#36389,#36390,
#36391,#36392,#36393,#36394,#36395,#36396,#36397,#36398,#36399,#36400,#36401,
#36402,#36403,#36404,#36405,#36406,#36407,#36408,#36409,#36410,#36411,#36412,
#36413,#36414,#36415,#36416,#36417,#36418,#36419,#36420,#36421,#36422,#36423,
#36424,#36425,#36426,#36427,#36428,#36429,#36430,#36431,#36432,#36433,#36434,
#36435,#36436,#36437,#36438,#36439,#36440,#36441,#36442,#36443,#36444,#36445,
#36446,#36447,#36448,#36449,#36450,#36451,#36452,#36453,#36454,#36455,#36456,
#36457,#36458,#36459,#36460,#36461,#36462,#36463,#36464,#36465,#36466,#36467,
#36468,#36469,#36470,#36471,#36472,#36473,#36474,#36475,#36476,#36477,#36478,
#36479,#36480,#36481,#36482,#36483,#36484,#36485,#36486,#36487,#36488,#36489,
#36490,#36491,#36492,#36493,#36494,#36495,#36496,#36497,#36498,#36499,#36500,
#36501,#36502,#36503,#36504,#36505,#36506,#36507,#36508,#36509,#36510,#36511,
#36512,#36513,#36514,#36515,#36516,#36517,#36518,#36519,#36520,#36521,#36522,
#36523,#36524,#36525,#36526,#36527,#36528,#36529,#36530,#36531,#36532,#36533,
#36534,#36535,#36536),.UNSPECIFIED.,.F.,.F.,(4,3,3,3,3,3,3,3,3,3,3,3,3,
3,3,3,3,3,3,3,3,3,3,3,3,3,3,3,3,3,3,3,3,3,3,3,3,3,3,3,3,3,3,3,3,3,3,3,3,
3,4),(30.4993214241099,30.589364887359,30.6765073736468,30.7680013253765,
30.8594952771061,30.9466072614862,31.0337024468151,31.1208004982627,31.2078937641911,
31.2950064517671,31.3468427748671,31.4339808001712,31.5211023922076,31.6082271424273,
31.6953472086888,31.7824866195326,31.8341902726282,31.9213169014601,32.0084269463445,
32.0955400358983,32.1826484052062,32.2697761653463,32.3215377703892,32.4086680911823,
32.4957818717525,32.5828987261604,32.6700108677988,32.7571423788036,32.8088852681502,
32.8960149192679,32.9831280267967,33.0702442097147,33.1573556823675,33.2444865341393,
33.2962327659112,33.3833626291845,33.4704759436101,33.5575923235023,33.6447039870287,
33.7318350185696,33.7835802636722,33.8707089656242,33.9578211205362,34.0449363548941,
34.1320468835505,34.2191768065887,34.2709277614332,34.3584567439305,34.4459664831206,
34.5334668399684,34.5575191894877),.UNSPECIFIED.);
#250=B_SPLINE_CURVE_WITH_KNOTS('',3,(#36537,#36538,#36539,#36540,#36541,
#36542,#36543,#36544,#36545),.UNSPECIFIED.,.F.,.F.,(4,1,1,1,1,1,4),(34.5575192147699,
34.7582752591942,35.2456227569552,35.7329702547162,36.2203177524772,36.7076652502382,
36.782513561854),.UNSPECIFIED.);
#251=B_SPLINE_CURVE_WITH_KNOTS('',3,(#36547,#36548,#36549,#36550,#36551,
#36552,#36553,#36554,#36555,#36556,#36557,#36558,#36559,#36560,#36561,#36562,
#36563,#36564,#36565,#36566,#36567,#36568,#36569,#36570,#36571,#36572,#36573,
#36574,#36575,#36576,#36577,#36578,#36579,#36580,#36581,#36582,#36583,#36584,
#36585,#36586,#36587,#36588,#36589,#36590,#36591,#36592,#36593,#36594,#36595,
#36596,#36597,#36598,#36599,#36600,#36601,#36602,#36603,#36604,#36605,#36606,
#36607,#36608,#36609,#36610,#36611,#36612,#36613,#36614,#36615,#36616,#36617,
#36618,#36619,#36620,#36621,#36622,#36623,#36624,#36625,#36626,#36627,#36628,
#36629,#36630,#36631),.UNSPECIFIED.,.F.,.F.,(4,3,3,3,3,3,3,3,3,3,3,3,3,
3,3,3,3,3,3,3,3,3,3,3,3,3,3,3,4),(34.5575191894877,34.6447569757657,34.7319918970944,
34.8192474416769,34.8682042325101,34.9553345524685,35.0424483321962,35.1295651857588,
35.2166773265522,35.3038088367198,35.3555517302711,35.4426813814716,35.5297944890805,
35.6169106720737,35.7040221447989,35.7911529966377,35.8428992280321,35.9300290910938,
36.0171424053112,36.1042587850018,36.191370448331,36.278501479683,36.3302467257931,
36.4173750047355,36.5086525326009,36.5957638112878,36.6828711022947,36.7699915625257,
36.7824851161968),.UNSPECIFIED.);
#252=B_SPLINE_CURVE_WITH_KNOTS('',3,(#36632,#36633,#36634,#36635,#36636,
#36637,#36638,#36639,#36640,#36641,#36642,#36643),.UNSPECIFIED.,.F.,.F.,
(4,1,1,1,1,1,1,1,1,4),(30.4992328073076,30.9694242504221,31.4567717481831,
31.9441192459441,32.4314667437051,32.9188142414661,33.4061617392271,33.8935092369881,
34.3808567347491,34.5575191593289),.UNSPECIFIED.);
#253=B_SPLINE_CURVE_WITH_KNOTS('',3,(#36649,#36650,#36651,#36652,#36653,
#36654,#36655,#36656,#36657,#36658,#36659,#36660,#36661,#36662,#36663,#36664,
#36665,#36666,#36667,#36668,#36669,#36670,#36671,#36672,#36673,#36674,#36675,
#36676,#36677,#36678,#36679,#36680,#36681,#36682,#36683,#36684,#36685,#36686,
#36687,#36688,#36689,#36690,#36691,#36692,#36693,#36694,#36695,#36696,#36697,
#36698,#36699,#36700,#36701,#36702,#36703,#36704,#36705,#36706,#36707,#36708,
#36709,#36710,#36711,#36712,#36713,#36714,#36715,#36716,#36717,#36718,#36719,
#36720,#36721,#36722,#36723,#36724,#36725,#36726,#36727,#36728,#36729,#36730,
#36731,#36732,#36733,#36734,#36735,#36736,#36737,#36738,#36739,#36740,#36741,
#36742,#36743,#36744,#36745,#36746,#36747,#36748,#36749,#36750,#36751,#36752,
#36753,#36754,#36755,#36756,#36757,#36758,#36759,#36760,#36761,#36762,#36763,
#36764,#36765,#36766,#36767,#36768,#36769,#36770,#36771,#36772,#36773,#36774,
#36775,#36776,#36777,#36778,#36779,#36780,#36781,#36782,#36783,#36784,#36785,
#36786,#36787,#36788,#36789,#36790,#36791,#36792,#36793,#36794,#36795,#36796,
#36797,#36798,#36799),.UNSPECIFIED.,.F.,.F.,(4,3,3,3,3,3,3,3,3,3,3,3,3,
3,3,3,3,3,3,3,3,3,3,3,3,3,3,3,3,3,3,3,3,3,3,3,3,3,3,3,3,3,3,3,3,3,3,3,3,
3,4),(24.2156474862923,24.3000483267107,24.3845029110786,24.4690844734779,
24.5239778062131,24.6055741796599,24.6870642443222,24.7684687650885,24.8498084045712,
24.9311114331561,25.0123964584347,25.0936820583996,25.174986810145,25.2563827962254,
25.337824621091,25.4194048181542,25.4986728017351,25.5832623133344,25.6677481822996,
25.7521477829318,25.836478417448,25.9207557824206,26.0050040171561,26.0892387031326,
26.1734754092372,26.2577612684093,26.3420733549027,26.426466141403,26.4733677972571,
26.558092298325,26.6427552017968,26.7273710330641,26.8119574560143,26.8965425130992,
26.9607152950181,27.0519442316041,27.1432666559618,27.2346896336238,27.3261417991208,
27.4176104484587,27.4480627927791,27.532586803755,27.6170657800487,27.7015239814603,
27.7859674988434,27.8704340010683,27.9354102905401,28.0240768753705,28.1127462609405,
28.2014356078663,28.2743338823081),.UNSPECIFIED.);
#254=B_SPLINE_CURVE_WITH_KNOTS('',3,(#36800,#36801,#36802,#36803,#36804,
#36805,#36806,#36807,#36808,#36809,#36810,#36811,#36812,#36813,#36814,#36815,
#36816,#36817,#36818,#36819,#36820,#36821,#36822,#36823,#36824,#36825,#36826,
#36827,#36828,#36829,#36830,#36831,#36832,#36833,#36834,#36835,#36836,#36837,
#36838,#36839,#36840,#36841,#36842,#36843,#36844,#36845,#36846,#36847,#36848,
#36849,#36850,#36851,#36852,#36853,#36854,#36855,#36856,#36857,#36858,#36859,
#36860,#36861,#36862,#36863,#36864,#36865,#36866,#36867,#36868,#36869,#36870,
#36871,#36872,#36873,#36874,#36875,#36876,#36877,#36878,#36879,#36880,#36881,
#36882,#36883,#36884),.UNSPECIFIED.,.F.,.F.,(4,3,3,3,3,3,3,3,3,3,3,3,3,
3,3,3,3,3,3,3,3,3,3,3,3,3,3,3,4),(28.2743338824266,28.3664532240664,28.4227577883011,
28.5092520935557,28.5957221727376,28.6821896165034,28.7686504765288,28.8551332349923,
28.9101052860621,28.9974342563849,29.084749014768,29.1720683332772,29.2593832734799,
29.3467162971122,29.3974527838231,29.4845626300906,29.5716559384561,29.6587525257064,
29.7458445655353,29.8329564077084,29.8848002815841,29.9719013840595,30.0589854167832,
30.1460720162916,30.2331536875928,30.3202546601054,30.3721477793451,30.459306450247,
30.4993214241099),.UNSPECIFIED.);
#255=B_SPLINE_CURVE_WITH_KNOTS('',3,(#36886,#36887,#36888,#36889,#36890,
#36891,#36892,#36893),.UNSPECIFIED.,.F.,.F.,(4,1,1,1,1,4),(28.2743353147298,
29.0200342593781,29.5073817571391,29.9947292549001,30.4820767526611,30.4992328073076),
 .UNSPECIFIED.);
#256=B_SPLINE_CURVE_WITH_KNOTS('',3,(#36894,#36895,#36896,#36897,#36898,
#36899,#36900,#36901,#36902,#36903,#36904,#36905,#36906,#36907,#36908,#36909,
#36910,#36911,#36912,#36913,#36914,#36915,#36916,#36917,#36918,#36919,#36920,
#36921,#36922,#36923,#36924,#36925,#36926,#36927,#36928,#36929,#36930,#36931,
#36932,#36933,#36934,#36935,#36936,#36937,#36938,#36939,#36940,#36941,#36942,
#36943,#36944,#36945,#36946,#36947,#36948,#36949,#36950,#36951,#36952,#36953,
#36954,#36955,#36956,#36957,#36958,#36959,#36960,#36961,#36962,#36963,#36964,
#36965,#36966,#36967,#36968,#36969,#36970,#36971,#36972,#36973,#36974,#36975,
#36976,#36977,#36978,#36979,#36980,#36981,#36982,#36983,#36984,#36985,#36986,
#36987,#36988,#36989,#36990,#36991,#36992,#36993,#36994,#36995,#36996,#36997,
#36998,#36999,#37000,#37001,#37002,#37003,#37004,#37005,#37006,#37007,#37008,
#37009,#37010,#37011,#37012,#37013,#37014,#37015,#37016,#37017,#37018,#37019,
#37020,#37021,#37022,#37023,#37024,#37025,#37026,#37027,#37028,#37029,#37030,
#37031,#37032,#37033,#37034,#37035,#37036,#37037,#37038,#37039,#37040,#37041),
 .UNSPECIFIED.,.F.,.F.,(4,3,3,3,3,3,3,3,3,3,3,3,3,3,3,3,3,3,3,3,3,3,3,3,
3,3,3,3,3,3,3,3,3,3,3,3,3,3,3,3,3,3,3,3,3,3,3,3,3,4),(24.2161265625725,
24.304879340127,24.3936266169366,24.4823579099005,24.57107729379,24.6339067795291,
24.7183716294415,24.8028157469338,24.887276430042,24.9717432184832,25.0562660667606,
25.1212542772901,25.2127216661248,25.304178010292,25.3955797066455,25.4869204524289,
25.5781480948867,25.6086017750511,25.6931817036893,25.7777588769285,25.8623793056185,
25.9470206674601,26.0317405844674,26.0959492728121,26.1803442406883,26.2646718670788,
26.3489493912654,26.4331940089271,26.5174394793457,26.6016893548484,26.6859592070288,
26.7702646181268,26.8546699103581,26.9391302810329,27.0237153293478,27.0706442683341,
27.1522405465237,27.2337305154638,27.3151349401118,27.3964744831466,27.4777774150383,
27.5590623434471,27.6403478464199,27.7216525011054,27.8030483905001,27.8844901186951,
27.9660702200751,28.0453392638561,28.1696765530861,28.2743338823081),
 .UNSPECIFIED.);
#257=B_SPLINE_CURVE_WITH_KNOTS('',3,(#37047,#37048,#37049,#37050,#37051,
#37052,#37053,#37054,#37055,#37056,#37057,#37058,#37059,#37060,#37061,#37062,
#37063,#37064,#37065,#37066,#37067,#37068,#37069,#37070,#37071,#37072,#37073,
#37074,#37075,#37076,#37077,#37078,#37079,#37080,#37081,#37082,#37083,#37084,
#37085,#37086,#37087,#37088,#37089,#37090,#37091,#37092,#37093,#37094,#37095,
#37096,#37097,#37098,#37099,#37100,#37101,#37102,#37103,#37104,#37105,#37106,
#37107,#37108,#37109,#37110,#37111,#37112,#37113,#37114,#37115,#37116,#37117,
#37118,#37119,#37120,#37121,#37122,#37123,#37124,#37125,#37126,#37127,#37128,
#37129,#37130,#37131),.UNSPECIFIED.,.F.,.F.,(4,3,3,3,3,3,3,3,3,3,3,3,3,
3,3,3,3,3,3,3,3,3,3,3,3,3,3,3,4),(15.7079632709821,15.7983391757108,15.861651819831,
15.9487473765214,16.0358259589805,16.1229073061607,16.2099838502341,16.2970799349332,
16.348999317592,16.4361366999986,16.523257608915,16.6103816220701,16.6975009223997,
16.7846395292193,16.836346815353,16.923477639889,17.010591951935,17.0977093744499,
17.1848221036438,17.2719542272672,17.323694313114,17.4108212348644,17.4979315648647,
17.5850449249431,17.6721535558284,17.7592815613529,17.811041810875,17.8981734346075,
17.932952833811),.UNSPECIFIED.);
#258=B_SPLINE_CURVE_WITH_KNOTS('',3,(#37133,#37134,#37135,#37136,#37137,
#37138),.UNSPECIFIED.,.F.,.F.,(4,1,1,4),(14.399609326548,14.886956824309,
15.37430432207,15.707963267949),.UNSPECIFIED.);
#259=B_SPLINE_CURVE_WITH_KNOTS('',3,(#37142,#37143,#37144,#37145,#37146,
#37147,#37148,#37149,#37150,#37151,#37152,#37153,#37154,#37155,#37156,#37157,
#37158,#37159,#37160,#37161,#37162,#37163,#37164,#37165,#37166,#37167,#37168,
#37169,#37170,#37171,#37172,#37173,#37174,#37175,#37176,#37177,#37178,#37179,
#37180,#37181,#37182,#37183,#37184,#37185,#37186,#37187,#37188,#37189,#37190,
#37191,#37192,#37193,#37194,#37195,#37196,#37197,#37198,#37199,#37200,#37201,
#37202,#37203,#37204,#37205,#37206,#37207,#37208),.UNSPECIFIED.,.F.,.F.,
(4,3,3,3,3,3,3,3,3,3,3,3,3,3,3,3,3,3,3,3,3,3,4),(13.8747245557601,13.9615196181783,
14.0483128516542,14.1350984649827,14.2219050359775,14.2896803532321,14.3768111748519,
14.4639254839518,14.5510429035049,14.638155629735,14.7252877504178,14.7770278509931,
14.864154772311,14.9512651018674,15.0383784614888,15.1254870919108,15.2126150969663,
15.2643753487541,15.3512430161605,15.4404230791076,15.5272738475405,15.6176185577448,
15.707963267949),.UNSPECIFIED.);
#260=B_SPLINE_CURVE_WITH_KNOTS('',3,(#37209,#37210,#37211,#37212,#37213,
#37214,#37215,#37216,#37217),.UNSPECIFIED.,.F.,.F.,(4,1,1,1,1,1,4),(15.707963267949,
15.7517228465151,16.2390703442761,16.7264178420371,17.2137653397981,17.7011128375591,
17.9329414836179),.UNSPECIFIED.);
#261=B_SPLINE_CURVE_WITH_KNOTS('',3,(#37223,#37224,#37225,#37226,#37227,
#37228),.UNSPECIFIED.,.F.,.F.,(4,1,1,4),(36.7825135685384,37.1950127479992,
37.6823602457602,38.1697077435212),.UNSPECIFIED.);
#262=B_SPLINE_CURVE_WITH_KNOTS('',3,(#37231,#37232,#37233,#37234,#37235,
#37236,#37237,#37238,#37239,#37240,#37241,#37242,#37243,#37244,#37245,#37246,
#37247,#37248,#37249,#37250,#37251,#37252,#37253,#37254,#37255,#37256,#37257,
#37258,#37259,#37260,#37261,#37262,#37263,#37264,#37265,#37266,#37267,#37268,
#37269,#37270,#37271,#37272,#37273,#37274,#37275,#37276,#37277,#37278,#37279,
#37280,#37281,#37282,#37283,#37284,#37285,#37286,#37287,#37288,#37289,#37290,
#37291,#37292,#37293,#37294,#37295,#37296,#37297,#37298,#37299,#37300,#37301,
#37302,#37303),.UNSPECIFIED.,.F.,.F.,(4,3,3,3,3,3,3,3,3,3,3,3,3,3,3,3,3,
3,3,3,3,3,3,3,4),(36.7824851168753,36.8175942235541,36.9047259024205,36.9918410382111,
37.0789592304617,37.1660726969111,37.2532055011074,37.3049417213151,37.3920685401476,
37.4791788111556,37.5662921786384,37.6534008545103,37.7405289626034,37.7922892190761,
37.8794201719593,37.966534565058,38.0536519969681,38.1407646949544,38.2278967250119,
38.2796367168371,38.3664398085489,38.4532349861649,38.5400191597449,38.6268188966943,
38.6945925143091),.UNSPECIFIED.);
#263=B_SPLINE_CURVE_WITH_KNOTS('',3,(#37309,#37310,#37311,#37312,#37313,
#37314,#37315,#37316,#37317,#37318,#37319,#37320,#37321,#37322,#37323,#37324,
#37325,#37326,#37327,#37328,#37329,#37330,#37331,#37332,#37333,#37334,#37335,
#37336,#37337,#37338,#37339,#37340,#37341,#37342,#37343,#37344,#37345,#37346,
#37347,#37348,#37349,#37350,#37351,#37352,#37353,#37354,#37355,#37356,#37357,
#37358,#37359,#37360,#37361,#37362,#37363,#37364,#37365,#37366,#37367,#37368,
#37369,#37370,#37371,#37372,#37373,#37374,#37375,#37376,#37377,#37378,#37379,
#37380,#37381,#37382,#37383,#37384,#37385,#37386,#37387,#37388,#37389,#37390,
#37391,#37392,#37393,#37394,#37395,#37396,#37397,#37398,#37399,#37400,#37401,
#37402,#37403,#37404,#37405,#37406,#37407,#37408,#37409,#37410,#37411,#37412,
#37413,#37414,#37415,#37416,#37417,#37418,#37419,#37420,#37421,#37422,#37423,
#37424,#37425,#37426,#37427,#37428,#37429,#37430,#37431,#37432,#37433,#37434,
#37435,#37436,#37437,#37438,#37439,#37440,#37441,#37442,#37443,#37444,#37445,
#37446,#37447,#37448,#37449,#37450,#37451,#37452,#37453,#37454,#37455,#37456,
#37457,#37458,#37459),.UNSPECIFIED.,.F.,.F.,(4,3,3,3,3,3,3,3,3,3,3,3,3,
3,3,3,3,3,3,3,3,3,3,3,3,3,3,3,3,3,3,3,3,3,3,3,3,3,3,3,3,3,3,3,3,3,3,3,3,
3,4),(30.4993214304177,30.5893648920898,30.6765072859223,30.7680012815142,
30.8594952771061,30.9466073231606,31.0337025710101,31.1208006856437,31.2078940149848,
31.2950067657722,31.3468427748671,31.4339807679861,31.5211023274172,31.6082270447182,
31.6953470779628,31.7824864559265,31.8341902726281,31.9213169142658,32.0084269721101,
32.0955400747291,32.1826484571305,32.2697762302935,32.3215377703891,32.4086680878499,
32.4957818650579,32.5828987160914,32.6700108543567,32.75714236202,32.8088852681501,
32.8960149195982,32.9831280274467,33.0702442106651,33.1573556836068,33.2444865356467,
33.2962327659111,33.3833626283388,33.4704759419317,33.5575923210181,33.6447039837563,
33.7318350145424,33.7835802636721,33.8707089685104,33.9578211263054,34.0449363635137,
34.1320468949955,34.2191768207951,34.2709277614331,34.3584567371214,34.4459664694995,
34.5334668195807,34.5575191894877),.UNSPECIFIED.);
#264=B_SPLINE_CURVE_WITH_KNOTS('',3,(#37460,#37461,#37462,#37463,#37464,
#37465,#37466,#37467,#37468),.UNSPECIFIED.,.F.,.F.,(4,1,1,1,1,1,4),(34.5575192147677,
34.7582752591941,35.2456227569552,35.7329702547162,36.2203177524772,36.7076652502382,
36.7825135685384),.UNSPECIFIED.);
#265=B_SPLINE_CURVE_WITH_KNOTS('',3,(#37470,#37471,#37472,#37473,#37474,
#37475,#37476,#37477,#37478,#37479,#37480,#37481,#37482,#37483,#37484,#37485,
#37486,#37487,#37488,#37489,#37490,#37491,#37492,#37493,#37494,#37495,#37496,
#37497,#37498,#37499,#37500,#37501,#37502,#37503,#37504,#37505,#37506,#37507,
#37508,#37509,#37510,#37511,#37512,#37513,#37514,#37515,#37516,#37517,#37518,
#37519,#37520,#37521,#37522,#37523,#37524,#37525,#37526,#37527,#37528,#37529,
#37530,#37531,#37532,#37533,#37534,#37535,#37536,#37537,#37538,#37539,#37540,
#37541,#37542,#37543,#37544,#37545,#37546,#37547,#37548,#37549,#37550,#37551,
#37552,#37553,#37554),.UNSPECIFIED.,.F.,.F.,(4,3,3,3,3,3,3,3,3,3,3,3,3,
3,3,3,3,3,3,3,3,3,3,3,3,3,3,3,4),(34.5575191894877,34.6447569868975,34.7319919193617,
34.8192474749927,34.8682042325101,34.9553345482705,35.0424483237626,35.1295651730742,
35.2166773096183,35.3038088155763,35.3555517302711,35.4426813818879,35.5297944898996,
35.6169106732714,35.7040221463605,35.7911529985374,35.8428992280321,35.9300290900273,
36.0171424031941,36.1042587818684,36.1913704442032,36.2785014746032,36.3302467257931,
36.4173750083753,36.5086525355003,36.5957638177863,36.6828711123603,36.7699915760908,
36.7824851168753),.UNSPECIFIED.);
#266=B_SPLINE_CURVE_WITH_KNOTS('',3,(#37555,#37556,#37557,#37558,#37559,
#37560,#37561,#37562,#37563,#37564,#37565,#37566),.UNSPECIFIED.,.F.,.F.,
(4,1,1,1,1,1,1,1,1,4),(30.4992330148162,30.9694242504221,31.4567717481831,
31.9441192459441,32.4314667437051,32.9188142414661,33.4061617392271,33.8935092369881,
34.3808567347491,34.5575191593334),.UNSPECIFIED.);
#267=B_SPLINE_CURVE_WITH_KNOTS('',3,(#37572,#37573,#37574,#37575,#37576,
#37577,#37578,#37579,#37580,#37581,#37582,#37583,#37584,#37585,#37586,#37587,
#37588,#37589,#37590,#37591,#37592,#37593,#37594,#37595,#37596,#37597,#37598,
#37599,#37600,#37601,#37602,#37603,#37604,#37605,#37606,#37607,#37608,#37609,
#37610,#37611,#37612,#37613,#37614,#37615,#37616,#37617,#37618,#37619,#37620,
#37621,#37622,#37623,#37624,#37625,#37626,#37627,#37628,#37629,#37630,#37631,
#37632,#37633,#37634,#37635,#37636,#37637,#37638,#37639,#37640,#37641,#37642,
#37643,#37644,#37645,#37646,#37647,#37648,#37649,#37650,#37651,#37652,#37653,
#37654,#37655,#37656,#37657,#37658,#37659,#37660,#37661,#37662,#37663,#37664,
#37665,#37666,#37667,#37668,#37669,#37670,#37671,#37672,#37673,#37674,#37675,
#37676,#37677,#37678,#37679,#37680,#37681,#37682,#37683,#37684,#37685,#37686,
#37687,#37688,#37689,#37690,#37691,#37692,#37693,#37694,#37695,#37696,#37697,
#37698,#37699,#37700,#37701,#37702,#37703,#37704,#37705,#37706,#37707,#37708,
#37709,#37710,#37711,#37712,#37713,#37714,#37715,#37716,#37717,#37718,#37719,
#37720,#37721,#37722),.UNSPECIFIED.,.F.,.F.,(4,3,3,3,3,3,3,3,3,3,3,3,3,
3,3,3,3,3,3,3,3,3,3,3,3,3,3,3,3,3,3,3,3,3,3,3,3,3,3,3,3,3,3,3,3,3,3,3,3,
3,4),(24.2156473321997,24.3000481377873,24.3845026911335,24.469084228759,
24.5239778062131,24.605573799559,24.687063482264,24.7684676194937,24.8498068741228,
24.931109516876,25.0123941556188,25.0936793685597,25.1749837330098,25.2563793332889,
25.3378207724143,25.4194005876772,25.4986728017351,25.583262289203,25.6677481290383,
25.7521476956501,25.8364782913607,25.9207556105826,26.0050037953159,26.0892384271216,
26.1734750749651,26.2577608699837,26.3420728889482,26.4264656031797,26.4733677972571,
26.5580943048163,26.642759224378,26.727377075819,26.8119655200819,26.8965525888317,
26.9607152950181,27.051939514377,27.1432570572615,27.234675022306,27.3261221417869,
27.4175857805144,27.4480627927791,27.5325902280114,27.617072650843,27.7015343147517,
27.7859813021922,27.8704512660146,27.9354102905401,28.0240739238239,28.1127403128143,
28.2014266288529,28.2743338823081),.UNSPECIFIED.);
#268=B_SPLINE_CURVE_WITH_KNOTS('',3,(#37723,#37724,#37725,#37726,#37727,
#37728,#37729,#37730,#37731,#37732,#37733,#37734,#37735,#37736,#37737,#37738,
#37739,#37740,#37741,#37742,#37743,#37744,#37745,#37746,#37747,#37748,#37749,
#37750,#37751,#37752,#37753,#37754,#37755,#37756,#37757,#37758,#37759,#37760,
#37761,#37762,#37763,#37764,#37765,#37766,#37767,#37768,#37769,#37770,#37771,
#37772,#37773,#37774,#37775,#37776,#37777,#37778,#37779,#37780,#37781,#37782,
#37783,#37784,#37785,#37786,#37787,#37788,#37789,#37790,#37791,#37792,#37793,
#37794,#37795,#37796,#37797,#37798,#37799,#37800,#37801,#37802,#37803,#37804,
#37805,#37806,#37807),.UNSPECIFIED.,.F.,.F.,(4,3,3,3,3,3,3,3,3,3,3,3,3,
3,3,3,3,3,3,3,3,3,3,3,3,3,3,3,4),(28.2743338824266,28.3664499676938,28.4227577883011,
28.5092534192787,28.5957248380328,28.6821936309558,28.768655843137,28.8551399477051,
28.9101052860621,28.9974337506621,29.0847479974582,29.1720668007956,29.2593812251369,
29.3467137364858,29.3974527838231,29.4845627017913,29.5716560821199,29.658752741023,
29.7458448521569,29.8329567644714,29.8848002815841,29.9719014591824,30.0589855683635,
30.1460722455977,30.2331539951606,30.3202550460865,30.3721477793451,30.459306360454,
30.4993214304177),.UNSPECIFIED.);
#269=B_SPLINE_CURVE_WITH_KNOTS('',3,(#37809,#37810,#37811,#37812,#37813,
#37814,#37815,#37816),.UNSPECIFIED.,.F.,.F.,(4,1,1,1,1,4),(28.2743353127056,
29.0200342593781,29.5073817571391,29.9947292549001,30.4820767526611,30.4992330148162),
 .UNSPECIFIED.);
#270=B_SPLINE_CURVE_WITH_KNOTS('',3,(#37817,#37818,#37819,#37820,#37821,
#37822,#37823,#37824,#37825,#37826,#37827,#37828,#37829,#37830,#37831,#37832,
#37833,#37834,#37835,#37836,#37837,#37838,#37839,#37840,#37841,#37842,#37843,
#37844,#37845,#37846,#37847,#37848,#37849,#37850,#37851,#37852,#37853,#37854,
#37855,#37856,#37857,#37858,#37859,#37860,#37861,#37862,#37863,#37864,#37865,
#37866,#37867,#37868,#37869,#37870,#37871,#37872,#37873,#37874,#37875,#37876,
#37877,#37878,#37879,#37880,#37881,#37882,#37883,#37884,#37885,#37886,#37887,
#37888,#37889,#37890,#37891,#37892,#37893,#37894,#37895,#37896,#37897,#37898,
#37899,#37900,#37901,#37902,#37903,#37904,#37905,#37906,#37907,#37908,#37909,
#37910,#37911,#37912,#37913,#37914,#37915,#37916,#37917,#37918,#37919,#37920,
#37921,#37922,#37923,#37924,#37925,#37926,#37927,#37928,#37929,#37930,#37931,
#37932,#37933,#37934,#37935,#37936,#37937,#37938,#37939,#37940,#37941,#37942,
#37943,#37944,#37945,#37946,#37947,#37948,#37949,#37950,#37951,#37952,#37953,
#37954,#37955,#37956,#37957,#37958,#37959,#37960,#37961,#37962,#37963,#37964),
 .UNSPECIFIED.,.F.,.F.,(4,3,3,3,3,3,3,3,3,3,3,3,3,3,3,3,3,3,3,3,3,3,3,3,
3,3,3,3,3,3,3,3,3,3,3,3,3,3,3,3,3,3,3,3,3,3,3,3,3,4),(24.2161266164728,
24.3048755834868,24.3936190635417,24.482346583967,24.5710622783973,24.6339067795291,
24.7183759992437,24.8028244958566,24.8872895482853,24.9717606994971,25.0562878722159,
25.1212542772901,25.212715341686,25.3041653224886,25.3955607374181,25.486895306588,
25.578117015447,25.6086017750511,25.6931842451492,25.7777639703814,25.8623869523081,
25.9470308674618,26.0317533205491,26.0959492728121,26.1803441484525,26.2646716876325,
26.3489491297302,26.433193670525,26.5174390722406,26.6016888841523,26.6859586779554,
26.770264035995,26.8546692836303,26.9391296144661,27.0237146307952,27.0706442683341,
27.1522400678308,27.2337295557392,27.3151334973669,27.3964725557215,27.4777750017013,
27.5590594433115,27.640344458871,27.7216486258011,27.8030440293227,27.8844852717219,
27.9660648922686,28.0453392638561,28.1696867713369,28.2743338823081),
 .UNSPECIFIED.);
#271=B_SPLINE_CURVE_WITH_KNOTS('',3,(#37970,#37971,#37972,#37973,#37974,
#37975,#37976,#37977,#37978,#37979,#37980,#37981,#37982,#37983,#37984,#37985,
#37986,#37987,#37988,#37989,#37990,#37991,#37992,#37993,#37994,#37995,#37996,
#37997,#37998,#37999,#38000,#38001,#38002,#38003,#38004,#38005,#38006,#38007,
#38008,#38009,#38010,#38011,#38012,#38013,#38014,#38015,#38016,#38017,#38018,
#38019,#38020,#38021,#38022,#38023,#38024,#38025,#38026,#38027,#38028,#38029,
#38030,#38031,#38032,#38033,#38034,#38035,#38036,#38037,#38038,#38039,#38040,
#38041,#38042,#38043,#38044,#38045,#38046,#38047,#38048,#38049,#38050,#38051,
#38052,#38053,#38054),.UNSPECIFIED.,.F.,.F.,(4,3,3,3,3,3,3,3,3,3,3,3,3,
3,3,3,3,3,3,3,3,3,3,3,3,3,3,3,4),(15.7079632709815,15.7983388023486,15.861651819831,
15.9487475083028,16.0358262241585,16.122907705879,16.2099843848246,16.2970806037435,
16.348999317592,16.4361366409196,16.5232574899998,16.6103814427677,16.6975006825434,
16.784639229082,16.836346815353,16.9234776545726,17.010591981452,17.0977094188805,
17.1848221629971,17.2719543014269,17.323694313114,17.4108212370465,17.4979315692867,
17.5850449316704,17.6721535648928,17.7592815727833,17.811041810875,17.8981734291986,
17.9329528346437),.UNSPECIFIED.);
#272=B_SPLINE_CURVE_WITH_KNOTS('',3,(#38056,#38057,#38058,#38059,#38060,
#38061),.UNSPECIFIED.,.F.,.F.,(4,1,1,4),(14.399609326548,14.886956824309,
15.37430432207,15.707963267949),.UNSPECIFIED.);
#273=B_SPLINE_CURVE_WITH_KNOTS('',3,(#38065,#38066,#38067,#38068,#38069,
#38070,#38071,#38072,#38073,#38074,#38075,#38076,#38077,#38078,#38079,#38080,
#38081,#38082,#38083,#38084,#38085,#38086,#38087,#38088,#38089,#38090,#38091,
#38092,#38093,#38094,#38095,#38096,#38097,#38098,#38099,#38100,#38101,#38102,
#38103,#38104,#38105,#38106,#38107,#38108,#38109,#38110,#38111,#38112,#38113,
#38114,#38115,#38116,#38117,#38118,#38119,#38120,#38121,#38122,#38123,#38124,
#38125,#38126,#38127,#38128,#38129,#38130,#38131),.UNSPECIFIED.,.F.,.F.,
(4,3,3,3,3,3,3,3,3,3,3,3,3,3,3,3,3,3,3,3,3,3,4),(13.8747245557601,13.96151957655,
14.0483127680288,14.1350983392423,14.2219048683033,14.289680353232,14.3768111864995,
14.4639255073661,14.5510429387493,14.6381556768169,14.7252878092448,14.777027850993,
14.8641547740402,14.9512651053716,15.03837846682,15.1254870990942,15.2126151060248,
15.264375348754,15.3512430123807,15.4404230762728,15.5272738407879,15.6176185543684,
15.707963267949),.UNSPECIFIED.);
#274=B_SPLINE_CURVE_WITH_KNOTS('',3,(#38132,#38133,#38134,#38135,#38136,
#38137,#38138,#38139,#38140),.UNSPECIFIED.,.F.,.F.,(4,1,1,1,1,1,4),(15.707963267949,
15.751722846515,16.239070344276,16.7264178420371,17.2137653397981,17.7011128375591,
17.9329414843961),.UNSPECIFIED.);
#275=B_SPLINE_CURVE_WITH_KNOTS('',3,(#38146,#38147,#38148,#38149,#38150,
#38151,#38152,#38153),.UNSPECIFIED.,.F.,.F.,(4,1,1,1,1,4),(181.295997048056,
181.669120728045,182.667957178007,183.666793627969,184.665630077931,185.353966561798),
 .UNSPECIFIED.);
#276=B_SPLINE_CURVE_WITH_KNOTS('',3,(#38155,#38156,#38157,#38158,#38159),
 .UNSPECIFIED.,.F.,.F.,(4,1,4),(185.353966561798,185.664466527893,186.663302977854),
 .UNSPECIFIED.);
#277=B_SPLINE_CURVE_WITH_KNOTS('',3,(#38163,#38164,#38165,#38166,#38167,
#38168,#38169,#38170,#38171,#38172,#38173,#38174,#38175,#38176,#38177,#38178,
#38179,#38180,#38181,#38182,#38183,#38184,#38185,#38186,#38187,#38188,#38189,
#38190,#38191,#38192,#38193,#38194,#38195,#38196,#38197,#38198,#38199,#38200,
#38201,#38202,#38203,#38204,#38205,#38206,#38207,#38208,#38209,#38210,#38211,
#38212,#38213,#38214,#38215,#38216,#38217,#38218,#38219,#38220),
 .UNSPECIFIED.,.F.,.F.,(4,3,3,3,3,3,3,3,3,3,3,3,3,3,3,3,3,3,3,4),(185.353966561798,
185.451129858625,185.54817353966,185.645152137366,185.742096643968,185.839038006741,
185.9360686719,186.033145887057,186.130383559085,186.198496245335,186.297011795472,
186.395389344314,186.494243526173,186.592449207881,186.690623911412,186.788797212158,
186.888153608916,186.986470035736,187.086346417463,187.18622279919),
 .UNSPECIFIED.);
#278=B_SPLINE_CURVE_WITH_KNOTS('',3,(#38221,#38222,#38223,#38224,#38225,
#38226,#38227,#38228),.UNSPECIFIED.,.F.,.F.,(4,1,1,1,1,4),(181.297167488959,
182.203150445487,183.201986895449,184.200823345411,185.199659795373,185.353966561798),
 .UNSPECIFIED.);
#279=B_SPLINE_CURVE_WITH_KNOTS('',3,(#38234,#38235,#38236,#38237,#38238,
#38239,#38240,#38241,#38242,#38243,#38244,#38245,#38246,#38247,#38248,#38249,
#38250,#38251,#38252,#38253,#38254,#38255,#38256,#38257,#38258,#38259,#38260,
#38261,#38262,#38263,#38264,#38265,#38266,#38267,#38268,#38269,#38270,#38271,
#38272,#38273,#38274,#38275,#38276,#38277,#38278,#38279,#38280,#38281,#38282,
#38283,#38284,#38285,#38286,#38287,#38288,#38289,#38290,#38291,#38292,#38293,
#38294,#38295,#38296,#38297,#38298,#38299,#38300,#38301,#38302,#38303,#38304,
#38305,#38306,#38307,#38308,#38309,#38310,#38311,#38312,#38313,#38314,#38315,
#38316,#38317,#38318,#38319,#38320,#38321,#38322,#38323,#38324,#38325,#38326,
#38327,#38328,#38329,#38330,#38331,#38332,#38333,#38334,#38335,#38336,#38337,
#38338,#38339,#38340,#38341,#38342,#38343,#38344,#38345,#38346,#38347,#38348,
#38349,#38350,#38351,#38352,#38353,#38354,#38355,#38356,#38357),
 .UNSPECIFIED.,.F.,.F.,(4,3,3,3,3,3,3,3,3,3,3,3,3,3,3,3,3,3,3,3,3,3,3,3,
3,3,3,3,3,3,3,3,3,3,3,3,3,3,3,3,3,4),(175.013888595044,175.112152253394,
175.210394737751,175.308645521428,175.40699963151,175.505407688072,175.603986032395,
175.676102028274,175.774697491594,175.873152609552,175.973375843138,176.071652747408,
176.169896682952,176.268137135791,176.369837471402,176.468219314363,176.571578896299,
176.674938478236,176.773539089412,176.871999342765,176.972221290944,177.070503263901,
177.168752232521,177.266997676458,177.368691989393,177.467078669032,177.570426798615,
177.673774928198,177.772377752086,177.87084027796,177.971061665485,178.069346039596,
178.167597451745,178.265845378085,178.367536878104,178.465926110356,178.569268744258,
178.672611378159,178.782250156969,178.891545552981,179.000249474037,179.070781030164),
 .UNSPECIFIED.);
#280=B_SPLINE_CURVE_WITH_KNOTS('',3,(#38358,#38359,#38360,#38361,#38362,
#38363),.UNSPECIFIED.,.F.,.F.,(4,1,1,4),(179.070781254618,179.671447828121,
180.670284278083,181.295997048056),.UNSPECIFIED.);
#281=B_SPLINE_CURVE_WITH_KNOTS('',3,(#38365,#38366,#38367,#38368,#38369,
#38370,#38371),.UNSPECIFIED.,.F.,.F.,(4,1,1,1,4),(179.070781254618,179.206641095602,
180.205477545564,181.204313995525,181.297167488959),.UNSPECIFIED.);
#282=B_SPLINE_CURVE_WITH_KNOTS('',3,(#38372,#38373,#38374,#38375,#38376,
#38377,#38378,#38379),.UNSPECIFIED.,.F.,.F.,(4,1,1,1,1,4),(175.012544756164,
175.211295295754,176.210131745716,177.208968195678,178.20780464564,179.070781254618),
 .UNSPECIFIED.);
#283=B_SPLINE_CURVE_WITH_KNOTS('',3,(#38385,#38386,#38387,#38388,#38389,
#38390,#38391,#38392,#38393,#38394,#38395,#38396,#38397,#38398,#38399,#38400,
#38401,#38402,#38403,#38404,#38405,#38406,#38407,#38408,#38409,#38410,#38411,
#38412,#38413,#38414,#38415,#38416,#38417,#38418,#38419,#38420,#38421,#38422,
#38423,#38424,#38425,#38426,#38427,#38428,#38429,#38430,#38431,#38432,#38433,
#38434,#38435,#38436,#38437,#38438,#38439,#38440,#38441,#38442,#38443,#38444,
#38445,#38446,#38447,#38448,#38449,#38450,#38451,#38452,#38453,#38454,#38455,
#38456,#38457,#38458,#38459,#38460,#38461,#38462,#38463,#38464,#38465,#38466,
#38467,#38468,#38469,#38470,#38471,#38472,#38473,#38474,#38475,#38476,#38477,
#38478,#38479,#38480,#38481,#38482,#38483,#38484,#38485,#38486,#38487,#38488,
#38489,#38490,#38491,#38492,#38493,#38494,#38495,#38496,#38497,#38498,#38499,
#38500,#38501,#38502,#38503,#38504,#38505,#38506,#38507,#38508),
 .UNSPECIFIED.,.F.,.F.,(4,3,3,3,3,3,3,3,3,3,3,3,3,3,3,3,3,3,3,3,3,3,3,3,
3,3,3,3,3,3,3,3,3,3,3,3,3,3,3,3,3,4),(168.73049948352,168.829027726418,
168.927431036374,169.025741344548,169.124002438926,169.222243820297,169.320494962343,
169.418850307068,169.517260913146,169.615840311951,169.683083328503,169.781681404697,
169.880139138671,169.980361718645,170.078641227933,170.176887758804,170.275130793941,
170.376828040072,170.475212406819,170.578566092641,170.681919778464,170.780517924844,
170.878975728609,170.979198291086,171.077477868714,171.175724467241,171.273967569265,
171.375664734055,171.474049165113,171.57740269677,171.680756228426,171.779354490085,
171.877812410303,171.978034943814,172.076314639908,172.174561357392,172.272804578702,
172.374501603624,172.472886153556,172.576239415972,172.679592678388,172.787595947439),
 .UNSPECIFIED.);
#284=B_SPLINE_CURVE_WITH_KNOTS('',3,(#38509,#38510,#38511,#38512,#38513,
#38514,#38515,#38516,#38517,#38518,#38519,#38520,#38521,#38522,#38523,#38524,
#38525,#38526,#38527,#38528,#38529,#38530,#38531,#38532,#38533,#38534,#38535,
#38536,#38537,#38538,#38539,#38540,#38541,#38542,#38543,#38544,#38545,#38546,
#38547,#38548,#38549,#38550,#38551,#38552,#38553,#38554,#38555,#38556,#38557,
#38558,#38559,#38560,#38561,#38562,#38563,#38564,#38565,#38566,#38567,#38568,
#38569,#38570,#38571,#38572,#38573,#38574,#38575,#38576,#38577,#38578,#38579,
#38580,#38581),.UNSPECIFIED.,.F.,.F.,(4,3,3,3,3,3,3,3,3,3,3,3,3,3,3,3,3,
3,3,3,3,3,3,3,4),(172.787595947668,172.884841559506,172.984040005612,173.081071838667,
173.178059271087,173.275033215733,173.375882193887,173.472980628238,173.570144972561,
173.667458410759,173.67842912835,173.777027506202,173.875485539322,173.975708044196,
174.073987844422,174.172234662569,174.270477980966,174.372174880302,174.470559517526,
174.573912547919,174.677265578312,174.775844825957,174.874301063312,174.972645507633,
175.013888595044),.UNSPECIFIED.);
#285=B_SPLINE_CURVE_WITH_KNOTS('',3,(#38583,#38584,#38585,#38586,#38587,
#38588),.UNSPECIFIED.,.F.,.F.,(4,1,1,4),(172.787601414733,173.21362239583,
174.212458845792,175.012544756164),.UNSPECIFIED.);
#286=B_SPLINE_CURVE_WITH_KNOTS('',3,(#38589,#38590,#38591,#38592,#38593,
#38594,#38595,#38596,#38597,#38598,#38599,#38600,#38601,#38602,#38603,#38604,
#38605,#38606,#38607,#38608,#38609,#38610,#38611,#38612,#38613,#38614,#38615,
#38616,#38617,#38618,#38619,#38620,#38621,#38622,#38623,#38624,#38625,#38626,
#38627,#38628,#38629,#38630,#38631,#38632,#38633,#38634,#38635,#38636,#38637,
#38638,#38639,#38640,#38641,#38642,#38643,#38644,#38645,#38646,#38647,#38648,
#38649,#38650,#38651,#38652,#38653,#38654,#38655,#38656,#38657,#38658,#38659,
#38660,#38661,#38662,#38663,#38664,#38665,#38666,#38667,#38668,#38669,#38670,
#38671,#38672,#38673,#38674,#38675,#38676,#38677,#38678,#38679,#38680,#38681,
#38682,#38683,#38684,#38685,#38686,#38687,#38688,#38689,#38690,#38691,#38692,
#38693,#38694,#38695,#38696,#38697,#38698,#38699,#38700,#38701,#38702,#38703,
#38704,#38705,#38706,#38707,#38708,#38709,#38710,#38711,#38712),
 .UNSPECIFIED.,.F.,.F.,(4,3,3,3,3,3,3,3,3,3,3,3,3,3,3,3,3,3,3,3,3,3,3,3,
3,3,3,3,3,3,3,3,3,3,3,3,3,3,3,3,3,4),(168.73021503563,168.828460503106,
168.92680521135,169.025197844636,169.123767881175,169.218276595983,169.316874714603,
169.415332491002,169.51555506037,169.61383461178,169.71208118457,169.810324261369,
169.912021457513,170.010405864863,170.113759455404,170.217113045945,170.315711171922,
170.414168955614,170.514391523151,170.612671081646,170.710917661431,170.809160745123,
170.910857932819,171.009242346745,171.112595921326,171.215949495907,171.314547642583,
171.413005447132,171.513228009474,171.611507589065,171.709754189987,171.807997294831,
171.90969445759,172.008078892486,172.111432419178,172.214785945869,172.315617765289,
172.416285943601,172.51678187547,172.617176498695,172.717484580153,172.787595947439),
 .UNSPECIFIED.);
#287=B_SPLINE_CURVE_WITH_KNOTS('',3,(#38718,#38719,#38720,#38721,#38722,
#38723,#38724,#38725),.UNSPECIFIED.,.F.,.F.,(4,1,1,1,1,4),(162.446146668403,
162.691228178769,163.690064628731,164.688901078693,165.687737528655,166.504405682607),
 .UNSPECIFIED.);
#288=B_SPLINE_CURVE_WITH_KNOTS('',3,(#38726,#38727,#38728,#38729,#38730,
#38731,#38732,#38733,#38734,#38735,#38736,#38737,#38738,#38739,#38740,#38741,
#38742,#38743,#38744,#38745,#38746,#38747,#38748,#38749,#38750,#38751,#38752,
#38753,#38754,#38755,#38756,#38757,#38758,#38759,#38760,#38761,#38762,#38763,
#38764,#38765,#38766,#38767,#38768,#38769,#38770,#38771,#38772,#38773,#38774,
#38775,#38776,#38777,#38778,#38779,#38780,#38781,#38782,#38783,#38784,#38785,
#38786,#38787,#38788,#38789,#38790,#38791,#38792,#38793,#38794,#38795),
 .UNSPECIFIED.,.F.,.F.,(4,3,3,3,3,3,3,3,3,3,3,3,3,3,3,3,3,3,3,3,3,3,3,4),
(166.504410640259,166.652910770048,166.686573978617,166.78517209724,166.883629873641,
166.983852443008,167.08213199442,167.180378567212,167.278621644013,167.380318840155,
167.478703247507,167.582056838043,167.685410428579,167.784008554557,167.882466338249,
167.982688905786,168.080968464281,168.179215044066,168.277458127759,168.379155315454,
168.477539729381,168.580893303961,168.684246878541,168.73049948352),
 .UNSPECIFIED.);
#289=B_SPLINE_CURVE_WITH_KNOTS('',3,(#38797,#38798,#38799,#38800,#38801,
#38802,#38803,#38804,#38805,#38806,#38807,#38808,#38809,#38810,#38811,#38812,
#38813,#38814,#38815,#38816,#38817,#38818,#38819,#38820,#38821,#38822,#38823,
#38824,#38825,#38826,#38827,#38828,#38829,#38830,#38831,#38832,#38833,#38834,
#38835,#38836,#38837,#38838,#38839,#38840,#38841,#38842,#38843,#38844,#38845,
#38846,#38847,#38848,#38849,#38850,#38851,#38852,#38853,#38854,#38855,#38856,
#38857,#38858,#38859,#38860,#38861,#38862,#38863,#38864,#38865,#38866,#38867,
#38868,#38869),.UNSPECIFIED.,.F.,.F.,(4,3,3,3,3,3,3,3,3,3,3,3,3,3,3,3,3,
3,3,3,3,3,3,3,4),(166.504410640259,166.6019131263,166.699371433808,166.79681599036,
166.894277201722,166.991846173226,167.089478292235,167.187269535436,167.220603696059,
167.319201820914,167.417659603534,167.517882171345,167.616161728897,167.714408307787,
167.812651390635,167.914348579482,168.012732992696,168.116086569359,168.219440146021,
168.318036793105,168.421081353736,168.51941990506,168.617691685804,168.715928358201,
168.73021503563),.UNSPECIFIED.);
#290=B_SPLINE_CURVE_WITH_KNOTS('',3,(#38870,#38871,#38872,#38873,#38874,
#38875,#38876,#38877,#38878,#38879,#38880,#38881,#38882,#38883,#38884,#38885,
#38886,#38887,#38888,#38889,#38890,#38891,#38892,#38893,#38894,#38895,#38896,
#38897,#38898,#38899,#38900,#38901,#38902,#38903,#38904,#38905,#38906,#38907,
#38908,#38909,#38910,#38911,#38912,#38913,#38914,#38915,#38916,#38917,#38918,
#38919,#38920,#38921,#38922,#38923,#38924,#38925,#38926,#38927,#38928,#38929,
#38930,#38931,#38932,#38933,#38934,#38935,#38936,#38937,#38938,#38939,#38940,
#38941,#38942,#38943,#38944,#38945,#38946,#38947,#38948,#38949,#38950,#38951,
#38952,#38953,#38954,#38955,#38956,#38957,#38958,#38959,#38960,#38961,#38962,
#38963,#38964,#38965,#38966,#38967,#38968,#38969,#38970,#38971,#38972,#38973,
#38974,#38975,#38976,#38977,#38978,#38979,#38980,#38981,#38982,#38983,#38984,
#38985,#38986,#38987,#38988,#38989,#38990,#38991,#38992,#38993),
 .UNSPECIFIED.,.F.,.F.,(4,3,3,3,3,3,3,3,3,3,3,3,3,3,3,3,3,3,3,3,3,3,3,3,
3,3,3,3,3,3,3,3,3,3,3,3,3,3,3,3,3,4),(162.447662171796,162.545987468187,
162.644256962553,162.742500165391,162.840746554158,162.939093168736,163.037489137586,
163.136060795295,163.225257896212,163.323856021116,163.422313803793,163.522536371591,
163.62081592922,163.719062508196,163.817305591138,163.919002779897,164.017387193222,
164.120740769698,164.224094346174,164.322692471118,164.421150253833,164.521372821621,
164.619652379285,164.717898958294,164.816142041267,164.917839229984,165.016223643336,
165.119577219736,165.222930796135,165.321528921635,165.419986704909,165.520209272557,
165.618488830783,165.716735410353,165.814978493886,165.916675681939,166.015060095843,
166.11841367097,166.221767246097,166.344599874415,166.465474953167,166.504410639987),
 .UNSPECIFIED.);
#291=B_SPLINE_CURVE_WITH_KNOTS('',3,(#38999,#39000,#39001,#39002,#39003,
#39004,#39005,#39006,#39007,#39008,#39009,#39010,#39011,#39012,#39013,#39014,
#39015,#39016,#39017,#39018,#39019,#39020,#39021,#39022,#39023,#39024,#39025,
#39026,#39027,#39028,#39029,#39030,#39031,#39032,#39033,#39034,#39035,#39036,
#39037,#39038,#39039,#39040,#39041,#39042,#39043,#39044,#39045,#39046,#39047,
#39048,#39049,#39050,#39051,#39052,#39053,#39054,#39055,#39056,#39057,#39058,
#39059,#39060,#39061,#39062,#39063,#39064,#39065,#39066,#39067,#39068,#39069,
#39070,#39071,#39072,#39073,#39074,#39075,#39076,#39077,#39078,#39079,#39080,
#39081,#39082,#39083,#39084,#39085,#39086,#39087,#39088,#39089,#39090,#39091,
#39092,#39093,#39094,#39095,#39096,#39097,#39098,#39099,#39100,#39101,#39102,
#39103,#39104,#39105,#39106,#39107,#39108,#39109,#39110,#39111,#39112,#39113,
#39114,#39115,#39116,#39117,#39118,#39119,#39120,#39121,#39122,#39123,#39124,
#39125),.UNSPECIFIED.,.F.,.F.,(4,3,3,3,3,3,3,3,3,3,3,3,3,3,3,3,3,3,3,3,
3,3,3,3,3,3,3,3,3,3,3,3,3,3,3,3,3,3,3,3,3,3,4),(156.163987530313,156.262228574752,
156.360486836606,156.458853630025,156.557282386566,156.655872483791,156.698209478998,
156.796807604012,156.895265386799,156.995487954569,157.093767512308,157.192014091391,
157.29025717444,157.39195436307,157.490338776499,157.593692352729,157.69704592896,
157.795644053952,157.894101836717,157.994324404493,158.092603962209,158.190850541271,
158.289093624298,158.390790812954,158.489175226362,158.592528802642,158.695882378922,
158.794480503912,158.892938286675,158.993160854451,159.091440412165,159.189686991224,
159.287930074248,159.389627262907,159.488011676312,159.591365252598,159.694718828884,
159.797216560019,159.903218753284,160.005303397591,160.107256278835,160.209067828953,
160.22122533308),.UNSPECIFIED.);
#292=B_SPLINE_CURVE_WITH_KNOTS('',3,(#39126,#39127,#39128,#39129,#39130,
#39131),.UNSPECIFIED.,.F.,.F.,(4,1,1,4),(160.221227414795,160.693555278846,
161.692391728808,162.446146668403),.UNSPECIFIED.);
#293=B_SPLINE_CURVE_WITH_KNOTS('',3,(#39133,#39134,#39135,#39136,#39137,
#39138,#39139,#39140,#39141,#39142,#39143,#39144,#39145,#39146,#39147,#39148,
#39149,#39150,#39151,#39152,#39153,#39154,#39155,#39156,#39157,#39158,#39159,
#39160,#39161,#39162,#39163,#39164,#39165,#39166,#39167,#39168,#39169,#39170,
#39171,#39172,#39173,#39174,#39175,#39176,#39177,#39178,#39179,#39180,#39181,
#39182,#39183,#39184,#39185,#39186,#39187,#39188,#39189,#39190,#39191,#39192,
#39193,#39194,#39195,#39196,#39197,#39198,#39199,#39200,#39201,#39202,#39203,
#39204,#39205),.UNSPECIFIED.,.F.,.F.,(4,3,3,3,3,3,3,3,3,3,3,3,3,3,3,3,3,
3,3,3,3,3,3,3,4),(160.22122533308,160.228748546326,160.327346671318,160.425804454083,
160.526027021859,160.624306579575,160.722553158637,160.820796241664,160.92249343032,
161.020877843728,161.124231420008,161.227584996288,161.326183121278,161.424640904041,
161.524863471817,161.623143029531,161.72138960859,161.819632691614,161.921329880273,
162.019714293678,162.123067869964,162.22642144625,162.325027406001,162.423481500101,
162.447662171796),.UNSPECIFIED.);
#294=B_SPLINE_CURVE_WITH_KNOTS('',3,(#39206,#39207,#39208,#39209,#39210,
#39211,#39212,#39213,#39214,#39215,#39216,#39217,#39218,#39219,#39220,#39221,
#39222,#39223,#39224,#39225,#39226,#39227,#39228,#39229,#39230,#39231,#39232,
#39233,#39234,#39235,#39236,#39237,#39238,#39239,#39240,#39241,#39242,#39243,
#39244,#39245,#39246,#39247,#39248,#39249,#39250,#39251,#39252,#39253,#39254,
#39255,#39256,#39257,#39258,#39259,#39260,#39261,#39262,#39263,#39264,#39265,
#39266,#39267,#39268,#39269,#39270,#39271,#39272,#39273,#39274,#39275,#39276,
#39277,#39278,#39279,#39280,#39281,#39282,#39283,#39284,#39285,#39286,#39287,
#39288,#39289,#39290,#39291,#39292,#39293,#39294,#39295,#39296,#39297,#39298,
#39299,#39300,#39301,#39302,#39303,#39304,#39305,#39306,#39307,#39308,#39309,
#39310,#39311,#39312,#39313,#39314,#39315,#39316,#39317,#39318,#39319,#39320,
#39321,#39322,#39323,#39324,#39325,#39326,#39327,#39328,#39329),
 .UNSPECIFIED.,.F.,.F.,(4,3,3,3,3,3,3,3,3,3,3,3,3,3,3,3,3,3,3,3,3,3,3,3,
3,3,3,3,3,3,3,3,3,3,3,3,3,3,3,3,3,4),(156.163531866271,156.233402746479,
156.332000871484,156.430458654262,156.530681222034,156.628960779764,156.727207358839,
156.825450441879,156.927147630519,157.025532043939,157.12888562019,157.23223919644,
157.330837321442,157.429295104218,157.529517671991,157.627797229718,157.72604380879,
157.824286891827,157.925984080471,158.024368493888,158.127722070145,158.231075646402,
158.329673771403,158.428131554177,158.528354121951,158.626633679676,158.724880258747,
158.823123341783,158.924820530428,159.023204943844,159.126558520104,159.229912096364,
159.328378576654,159.426704810661,159.526019875932,159.624169149678,159.722285836342,
159.820399593048,159.920606027993,160.018861091251,160.120043212039,160.221225332828),
 .UNSPECIFIED.);
#295=B_SPLINE_CURVE_WITH_KNOTS('',3,(#39335,#39336,#39337,#39338,#39339,
#39340,#39341,#39342),.UNSPECIFIED.,.F.,.F.,(4,1,1,1,1,4),(149.881541639708,
150.705190779227,151.704027229189,152.702863679151,153.701700129113,153.938039726867),
 .UNSPECIFIED.);
#296=B_SPLINE_CURVE_WITH_KNOTS('',3,(#39343,#39344,#39345,#39346,#39347,
#39348,#39349,#39350,#39351,#39352,#39353,#39354,#39355,#39356,#39357,#39358,
#39359,#39360,#39361,#39362,#39363,#39364,#39365,#39366,#39367,#39368,#39369,
#39370,#39371,#39372,#39373,#39374,#39375,#39376,#39377,#39378,#39379,#39380,
#39381,#39382,#39383,#39384,#39385,#39386,#39387,#39388,#39389,#39390,#39391,
#39392,#39393,#39394,#39395,#39396,#39397,#39398,#39399,#39400,#39401,#39402,
#39403,#39404,#39405,#39406,#39407,#39408,#39409,#39410,#39411,#39412),
 .UNSPECIFIED.,.F.,.F.,(4,3,3,3,3,3,3,3,3,3,3,3,3,3,3,3,3,3,3,3,3,3,3,4),
(153.9380400259,154.035163898234,154.132222574362,154.229246955324,154.326267897773,
154.423381488606,154.520541056366,154.617870832504,154.700536579074,154.799134704076,
154.897592486852,154.997815054625,155.096094612352,155.194341191424,155.292584274461,
155.394281463105,155.492665876523,155.596019452779,155.699373029036,155.797975862229,
155.896415143044,155.994759399118,156.093038592398,156.163987530313),
 .UNSPECIFIED.);
#297=B_SPLINE_CURVE_WITH_KNOTS('',3,(#39414,#39415,#39416,#39417,#39418,
#39419,#39420,#39421,#39422,#39423,#39424,#39425,#39426,#39427,#39428,#39429,
#39430,#39431,#39432,#39433,#39434,#39435,#39436,#39437,#39438,#39439,#39440,
#39441,#39442,#39443,#39444,#39445,#39446,#39447,#39448,#39449,#39450,#39451,
#39452,#39453,#39454,#39455,#39456,#39457,#39458,#39459,#39460,#39461,#39462,
#39463,#39464,#39465,#39466,#39467,#39468,#39469,#39470,#39471,#39472,#39473,
#39474,#39475,#39476,#39477,#39478,#39479,#39480,#39481,#39482,#39483),
 .UNSPECIFIED.,.F.,.F.,(4,3,3,3,3,3,3,3,3,3,3,3,3,3,3,3,3,3,3,3,3,3,3,4),
(153.938040202769,154.056659980237,154.176963650994,154.235729846555,154.334327971559,
154.432785754335,154.533008322108,154.631287879836,154.729534458909,154.827777541948,
154.92947473059,155.027859144009,155.131212720263,155.234566296517,155.333169148014,
155.431630381054,155.529972651705,155.628250049486,155.726492098718,155.824728281924,
155.923038846763,156.021391522228,156.119876942615,156.163531866271),
 .UNSPECIFIED.);
#298=B_SPLINE_CURVE_WITH_KNOTS('',3,(#39484,#39485,#39486,#39487,#39488,
#39489,#39490,#39491),.UNSPECIFIED.,.F.,.F.,(4,1,1,1,1,4),(149.880018430852,
150.240384046707,151.239220496669,152.238056946631,153.236893396593,153.9380400259),
 .UNSPECIFIED.);
#299=B_SPLINE_CURVE_WITH_KNOTS('',3,(#39497,#39498,#39499,#39500,#39501,
#39502,#39503,#39504,#39505,#39506,#39507,#39508,#39509,#39510,#39511,#39512,
#39513,#39514,#39515,#39516,#39517,#39518,#39519,#39520,#39521,#39522,#39523,
#39524,#39525,#39526,#39527,#39528,#39529,#39530,#39531,#39532,#39533,#39534,
#39535,#39536,#39537,#39538,#39539,#39540,#39541,#39542,#39543,#39544,#39545,
#39546,#39547,#39548,#39549,#39550,#39551,#39552,#39553,#39554,#39555,#39556,
#39557,#39558,#39559,#39560,#39561,#39562,#39563,#39564,#39565,#39566,#39567,
#39568,#39569,#39570,#39571,#39572,#39573,#39574,#39575,#39576,#39577,#39578,
#39579,#39580,#39581,#39582,#39583,#39584,#39585,#39586,#39587,#39588,#39589,
#39590,#39591,#39592,#39593,#39594,#39595,#39596,#39597,#39598,#39599,#39600,
#39601,#39602,#39603,#39604,#39605,#39606,#39607,#39608,#39609,#39610,#39611,
#39612,#39613,#39614,#39615,#39616,#39617,#39618,#39619,#39620,#39621,#39622,
#39623),.UNSPECIFIED.,.F.,.F.,(4,3,3,3,3,3,3,3,3,3,3,3,3,3,3,3,3,3,3,3,
3,3,3,3,3,3,3,3,3,3,3,3,3,3,3,3,3,3,3,3,3,3,4),(143.597018446188,143.695621188533,
143.713335629494,143.811933754498,143.910391537275,144.010614105047,144.108893662775,
144.207140241849,144.305383324887,144.40708051353,144.505464926948,144.608818503202,
144.712172079456,144.81077020446,144.909227987236,145.009450555009,145.107730112737,
145.20597669181,145.304219774849,145.405916963491,145.50430137691,145.607654953164,
145.711008529418,145.809606654422,145.908064437198,146.008287004971,146.106566562699,
146.204813141772,146.303056224811,146.404753413453,146.503137826872,146.606491403125,
146.709844979379,146.807643480436,146.905302408374,147.002849316603,147.100335701354,
147.197792033696,147.295248746519,147.392798083501,147.490396206244,147.588155506493,
147.65485471872),.UNSPECIFIED.);
#300=B_SPLINE_CURVE_WITH_KNOTS('',3,(#39624,#39625,#39626,#39627,#39628,
#39629,#39630),.UNSPECIFIED.,.F.,.F.,(4,1,1,1,4),(147.65485471872,147.708681429341,
148.707517879303,149.706354329265,149.881541639708),.UNSPECIFIED.);
#301=B_SPLINE_CURVE_WITH_KNOTS('',3,(#39632,#39633,#39634,#39635,#39636,
#39637),.UNSPECIFIED.,.F.,.F.,(4,1,1,4),(147.65485471872,148.242711146784,
149.241547596745,149.880018430852),.UNSPECIFIED.);
#302=B_SPLINE_CURVE_WITH_KNOTS('',3,(#39638,#39639,#39640,#39641,#39642,
#39643,#39644,#39645,#39646,#39647,#39648,#39649,#39650,#39651,#39652,#39653,
#39654,#39655,#39656,#39657,#39658,#39659,#39660,#39661,#39662,#39663,#39664,
#39665,#39666,#39667,#39668,#39669,#39670,#39671,#39672,#39673,#39674,#39675,
#39676,#39677,#39678,#39679,#39680,#39681,#39682,#39683,#39684,#39685,#39686,
#39687,#39688,#39689,#39690,#39691,#39692,#39693,#39694,#39695,#39696,#39697,
#39698,#39699,#39700,#39701,#39702,#39703,#39704,#39705,#39706,#39707,#39708,
#39709,#39710,#39711,#39712,#39713,#39714,#39715,#39716,#39717,#39718,#39719,
#39720,#39721,#39722,#39723,#39724,#39725,#39726,#39727,#39728,#39729,#39730,
#39731,#39732,#39733,#39734,#39735,#39736,#39737,#39738,#39739,#39740,#39741,
#39742,#39743,#39744,#39745,#39746,#39747,#39748,#39749,#39750,#39751,#39752,
#39753,#39754,#39755,#39756,#39757,#39758,#39759,#39760,#39761),
 .UNSPECIFIED.,.F.,.F.,(4,3,3,3,3,3,3,3,3,3,3,3,3,3,3,3,3,3,3,3,3,3,3,3,
3,3,3,3,3,3,3,3,3,3,3,3,3,3,3,3,3,4),(143.597933860091,143.696192254726,
143.794433309395,143.89268649678,143.991045284982,144.089461466197,144.188044027423,
144.247365346936,144.34596347194,144.444421254716,144.544643822489,144.642923380217,
144.741169959291,144.839413042329,144.941110230971,145.03949464439,145.142848220644,
145.246201796898,145.344799921902,145.443257704679,145.543480272451,145.64175983018,
145.740006409253,145.838249492291,145.939946680933,146.038331094352,146.141684670606,
146.24503824686,146.343636371864,146.442094154641,146.542316722413,146.640596280141,
146.738842859215,146.837085942254,146.938783130896,147.037167544314,147.140521120568,
147.243874696822,147.352569174393,147.460952550047,147.568802109383,147.654854305396),
 .UNSPECIFIED.);
#303=B_SPLINE_CURVE_WITH_KNOTS('',3,(#39767,#39768,#39769,#39770,#39771,
#39772,#39773,#39774,#39775,#39776,#39777,#39778,#39779,#39780,#39781,#39782,
#39783,#39784,#39785,#39786,#39787,#39788,#39789,#39790,#39791,#39792,#39793,
#39794,#39795,#39796,#39797,#39798,#39799,#39800,#39801,#39802,#39803,#39804,
#39805,#39806,#39807,#39808,#39809,#39810,#39811,#39812,#39813,#39814,#39815,
#39816,#39817,#39818,#39819,#39820,#39821,#39822,#39823,#39824,#39825,#39826,
#39827,#39828,#39829,#39830,#39831,#39832,#39833,#39834,#39835,#39836,#39837,
#39838,#39839,#39840,#39841,#39842,#39843,#39844,#39845,#39846,#39847,#39848,
#39849,#39850,#39851,#39852,#39853,#39854,#39855,#39856,#39857,#39858,#39859,
#39860,#39861,#39862,#39863,#39864,#39865,#39866,#39867,#39868,#39869,#39870,
#39871,#39872,#39873,#39874,#39875,#39876,#39877,#39878,#39879,#39880,#39881,
#39882,#39883,#39884,#39885,#39886,#39887,#39888,#39889,#39890),
 .UNSPECIFIED.,.F.,.F.,(4,3,3,3,3,3,3,3,3,3,3,3,3,3,3,3,3,3,3,3,3,3,3,3,
3,3,3,3,3,3,3,3,3,3,3,3,3,3,3,3,3,4),(137.314044031679,137.41561225619,
137.513996896003,137.617156912863,137.720316929723,137.818915054727,137.917372837504,
138.017595405276,138.115874963004,138.214121542078,138.312364625116,138.414061813758,
138.512446227177,138.61579980343,138.719153379684,138.817751504688,138.916209287464,
139.016431855237,139.114711412965,139.212957992039,139.311201075077,139.412898263719,
139.511282677138,139.614636253392,139.717989829646,139.81658795465,139.915045737427,
140.015268305199,140.113547862927,140.211794442001,140.310037525039,140.411734713682,
140.5101191271,140.613472703354,140.716826279608,140.815569227393,140.914173010821,
141.012667061739,141.111081830931,141.209449097701,141.307822396312,141.371669411541),
 .UNSPECIFIED.);
#304=B_SPLINE_CURVE_WITH_KNOTS('',3,(#39891,#39892,#39893,#39894,#39895,
#39896,#39897,#39898,#39899,#39900,#39901,#39902,#39903,#39904,#39905,#39906,
#39907,#39908,#39909,#39910,#39911,#39912,#39913,#39914,#39915,#39916,#39917,
#39918,#39919,#39920,#39921,#39922,#39923,#39924,#39925,#39926,#39927,#39928,
#39929,#39930,#39931,#39932,#39933,#39934,#39935,#39936,#39937,#39938,#39939,
#39940,#39941,#39942,#39943,#39944,#39945,#39946,#39947,#39948,#39949,#39950,
#39951,#39952,#39953,#39954,#39955,#39956,#39957),.UNSPECIFIED.,.F.,.F.,
(4,3,3,3,3,3,3,3,3,3,3,3,3,3,3,3,3,3,3,3,3,3,4),(141.371669411768,141.485016004535,
141.600339367052,141.71566272957,141.814260854574,141.91271863735,142.012941205123,
142.111220762851,142.209467341925,142.307710424963,142.409407613605,142.507792027024,
142.611145603278,142.714499179532,142.813105314799,142.911543009971,143.009885026333,
143.108160960057,143.206400336868,143.304679404108,143.402973649619,143.501391759057,
143.597018446188),.UNSPECIFIED.);
#305=B_SPLINE_CURVE_WITH_KNOTS('',3,(#39959,#39960,#39961,#39962,#39963,
#39964,#39965,#39966,#39967,#39968,#39969,#39970,#39971,#39972,#39973,#39974,
#39975,#39976,#39977,#39978,#39979,#39980,#39981,#39982,#39983,#39984,#39985,
#39986,#39987,#39988,#39989,#39990,#39991,#39992,#39993,#39994,#39995,#39996,
#39997,#39998,#39999,#40000,#40001,#40002,#40003,#40004,#40005,#40006,#40007,
#40008,#40009,#40010,#40011,#40012,#40013,#40014,#40015,#40016,#40017,#40018,
#40019,#40020,#40021,#40022,#40023,#40024,#40025,#40026,#40027,#40028),
 .UNSPECIFIED.,.F.,.F.,(4,3,3,3,3,3,3,3,3,3,3,3,3,3,3,3,3,3,3,3,3,3,3,4),
(141.371669411541,141.468831254161,141.566438903267,141.66339620349,141.760311911022,
141.857216996242,141.955335858935,142.052368429038,142.151030438025,142.249692447012,
142.348290572016,142.446748354792,142.546970922565,142.645250480293,142.743497059367,
142.841740142405,142.943437331047,143.041821744466,143.14517532072,143.248528896974,
143.347104955711,143.445558136395,143.543900701735,143.597933860091),
 .UNSPECIFIED.);
#306=B_SPLINE_CURVE_WITH_KNOTS('',3,(#40029,#40030,#40031,#40032,#40033,
#40034,#40035,#40036),.UNSPECIFIED.,.F.,.F.,(4,1,1,1,1,4),(137.314688012658,
138.254346647165,139.253183097127,140.252019547089,141.25085599705,141.371669411541),
 .UNSPECIFIED.);
#307=B_SPLINE_CURVE_WITH_KNOTS('',3,(#40042,#40043,#40044,#40045,#40046,
#40047,#40048,#40049,#40050,#40051,#40052,#40053,#40054,#40055,#40056,#40057,
#40058,#40059,#40060,#40061,#40062,#40063,#40064,#40065,#40066,#40067,#40068,
#40069,#40070,#40071,#40072,#40073,#40074,#40075,#40076,#40077,#40078,#40079,
#40080,#40081,#40082,#40083,#40084,#40085,#40086,#40087,#40088,#40089,#40090,
#40091,#40092,#40093,#40094,#40095,#40096,#40097,#40098,#40099,#40100,#40101,
#40102,#40103,#40104,#40105,#40106,#40107,#40108,#40109,#40110,#40111,#40112,
#40113,#40114,#40115,#40116,#40117,#40118,#40119,#40120,#40121,#40122,#40123,
#40124,#40125,#40126,#40127,#40128,#40129,#40130,#40131,#40132,#40133,#40134,
#40135,#40136,#40137,#40138,#40139,#40140,#40141,#40142,#40143,#40144,#40145,
#40146,#40147,#40148,#40149,#40150,#40151,#40152,#40153,#40154,#40155,#40156,
#40157,#40158,#40159,#40160,#40161,#40162,#40163,#40164,#40165),
 .UNSPECIFIED.,.F.,.F.,(4,3,3,3,3,3,3,3,3,3,3,3,3,3,3,3,3,3,3,3,3,3,3,3,
3,3,3,3,3,3,3,3,3,3,3,3,3,3,3,3,3,4),(131.031654909927,131.129931649269,
131.228177184675,131.326420997262,131.426640305434,131.525027337791,131.626162783871,
131.727298229951,131.825896354955,131.924354137731,132.024576705504,132.122856263232,
132.221102842306,132.319345925344,132.421043113987,132.519427527405,132.622781103659,
132.726134679913,132.824732804917,132.923190587693,133.023413155466,133.121692713194,
133.219939292268,133.318182375306,133.419879563948,133.518263977367,133.621617553621,
133.724971129875,133.823569254879,133.922027037655,134.022249605428,134.120529163156,
134.218775742229,134.317018825268,134.41871601391,134.517100427329,134.620454003583,
134.723807579837,134.8363385207,134.948409000642,135.059693750754,135.088484104126),
 .UNSPECIFIED.);
#308=B_SPLINE_CURVE_WITH_KNOTS('',3,(#40166,#40167,#40168,#40169,#40170,
#40171,#40172,#40173,#40174,#40175,#40176,#40177,#40178,#40179,#40180,#40181,
#40182,#40183,#40184,#40185,#40186,#40187,#40188,#40189,#40190,#40191,#40192,
#40193,#40194,#40195,#40196,#40197,#40198,#40199,#40200,#40201,#40202,#40203,
#40204,#40205,#40206,#40207,#40208,#40209,#40210,#40211,#40212,#40213,#40214,
#40215,#40216,#40217,#40218,#40219,#40220,#40221,#40222,#40223,#40224,#40225,
#40226,#40227,#40228,#40229,#40230,#40231,#40232,#40233,#40234,#40235),
 .UNSPECIFIED.,.F.,.F.,(4,3,3,3,3,3,3,3,3,3,3,3,3,3,3,3,3,3,3,3,3,3,3,4),
(135.088484104361,135.187254556185,135.286029876603,135.384838499173,135.483776463585,
135.582788468007,135.681976179005,135.722644029799,135.821242154803,135.919699937579,
136.019922505352,136.11820206308,136.216448642154,136.314691725192,136.416388913834,
136.514773327253,136.618126903507,136.721480479761,136.820067256337,136.918521077998,
137.017401816418,137.115677656305,137.214860843992,137.314044031679),
 .UNSPECIFIED.);
#309=B_SPLINE_CURVE_WITH_KNOTS('',3,(#40237,#40238,#40239,#40240,#40241,
#40242,#40243),.UNSPECIFIED.,.F.,.F.,(4,1,1,1,4),(135.088484104361,135.257837297279,
136.256673747241,137.255510197203,137.314688012658),.UNSPECIFIED.);
#310=B_SPLINE_CURVE_WITH_KNOTS('',3,(#40244,#40245,#40246,#40247,#40248,
#40249,#40250,#40251,#40252,#40253,#40254,#40255,#40256,#40257,#40258,#40259,
#40260,#40261,#40262,#40263,#40264,#40265,#40266,#40267,#40268,#40269,#40270,
#40271,#40272,#40273,#40274,#40275,#40276,#40277,#40278,#40279,#40280,#40281,
#40282,#40283,#40284,#40285,#40286,#40287,#40288,#40289,#40290,#40291,#40292,
#40293,#40294,#40295,#40296,#40297,#40298,#40299,#40300,#40301,#40302,#40303,
#40304,#40305,#40306,#40307,#40308,#40309,#40310,#40311,#40312,#40313,#40314,
#40315,#40316,#40317,#40318,#40319,#40320,#40321,#40322,#40323,#40324,#40325,
#40326,#40327,#40328,#40329,#40330,#40331,#40332,#40333,#40334,#40335,#40336,
#40337,#40338,#40339,#40340,#40341,#40342,#40343,#40344,#40345,#40346,#40347,
#40348,#40349,#40350,#40351,#40352,#40353,#40354,#40355,#40356,#40357,#40358,
#40359,#40360,#40361,#40362,#40363,#40364,#40365,#40366,#40367,#40368,#40369,
#40370),.UNSPECIFIED.,.F.,.F.,(4,3,3,3,3,3,3,3,3,3,3,3,3,3,3,3,3,3,3,3,
3,3,3,3,3,3,3,3,3,3,3,3,3,3,3,3,3,3,3,3,3,3,4),(131.030544881201,131.128979377099,
131.227573069973,131.262491497432,131.361089622436,131.459547405212,131.559769972985,
131.658049530713,131.756296109786,131.854539192825,131.956236381467,132.054620794886,
132.15797437114,132.261327947394,132.359926072398,132.458383855174,132.558606422947,
132.656885980675,132.755132559748,132.853375642787,132.955072831429,133.053457244848,
133.156810821101,133.260164397355,133.358762522359,133.457220305135,133.557442872908,
133.655722430636,133.753969009709,133.852212092748,133.95390928139,134.052293694809,
134.155647271063,134.259000847317,134.356128675187,134.453094160804,134.549968416923,
134.6467826177,134.743567858739,134.84039997176,134.937256811786,135.034231214226,
135.088484104361),.UNSPECIFIED.);
#311=B_SPLINE_CURVE_WITH_KNOTS('',3,(#40376,#40377,#40378,#40379,#40380,
#40381,#40382,#40383),.UNSPECIFIED.,.F.,.F.,(4,1,1,1,1,4),(124.748033420129,
125.73427953018,126.733115980142,127.731952430104,128.730788880066,128.805298797182),
 .UNSPECIFIED.);
#312=B_SPLINE_CURVE_WITH_KNOTS('',3,(#40384,#40385,#40386,#40387,#40388,
#40389,#40390,#40391,#40392,#40393,#40394,#40395,#40396,#40397,#40398,#40399,
#40400,#40401,#40402,#40403,#40404,#40405,#40406,#40407,#40408,#40409,#40410,
#40411,#40412,#40413,#40414,#40415,#40416,#40417,#40418,#40419,#40420,#40421,
#40422,#40423,#40424,#40425,#40426,#40427,#40428,#40429,#40430,#40431,#40432,
#40433,#40434,#40435,#40436,#40437,#40438,#40439,#40440,#40441,#40442,#40443,
#40444,#40445,#40446,#40447,#40448,#40449,#40450,#40451,#40452,#40453),
 .UNSPECIFIED.,.F.,.F.,(4,3,3,3,3,3,3,3,3,3,3,3,3,3,3,3,3,3,3,3,3,3,3,4),
(128.805298797182,128.902840431273,129.000250613517,129.097560812666,129.194818343698,
129.292053887497,129.389298094495,129.486642967568,129.584044330746,129.68160592498,
129.729625330028,129.828223455032,129.926681237808,130.026903805581,130.125183363309,
130.223429942382,130.321673025421,130.423370214063,130.521754627482,130.625108203735,
130.728461779989,130.827047027854,130.92935096889,131.031654909927),
 .UNSPECIFIED.);
#313=B_SPLINE_CURVE_WITH_KNOTS('',3,(#40455,#40456,#40457,#40458,#40459,
#40460,#40461,#40462,#40463,#40464,#40465,#40466,#40467,#40468,#40469,#40470,
#40471,#40472,#40473,#40474,#40475,#40476,#40477,#40478,#40479,#40480,#40481,
#40482,#40483,#40484,#40485,#40486,#40487,#40488,#40489,#40490,#40491,#40492,
#40493,#40494,#40495,#40496,#40497,#40498,#40499,#40500,#40501,#40502,#40503,
#40504,#40505,#40506,#40507,#40508,#40509,#40510,#40511,#40512,#40513,#40514,
#40515,#40516,#40517,#40518,#40519,#40520,#40521,#40522,#40523,#40524),
 .UNSPECIFIED.,.F.,.F.,(4,3,3,3,3,3,3,3,3,3,3,3,3,3,3,3,3,3,3,3,3,3,3,4),
(128.805299011162,128.910085619872,129.015255759152,129.120630109634,129.226318351048,
129.264818597508,129.363416722512,129.461874505289,129.562097073061,129.660376630789,
129.758623209863,129.856866292901,129.958563481543,130.056947894962,130.160301471216,
130.26365504747,130.36222548666,130.460667523607,130.5590108659,130.657285118185,
130.755545076202,130.853792579344,130.95210867263,131.030544881201),
 .UNSPECIFIED.);
#314=B_SPLINE_CURVE_WITH_KNOTS('',3,(#40525,#40526,#40527,#40528,#40529,
#40530,#40531,#40532),.UNSPECIFIED.,.F.,.F.,(4,1,1,1,1,4),(124.748072377546,
125.26947279766,126.268309247622,127.267145697584,128.265982147546,128.805298797182),
 .UNSPECIFIED.);
#315=B_SPLINE_CURVE_WITH_KNOTS('',3,(#40538,#40539,#40540,#40541,#40542,
#40543,#40544,#40545,#40546,#40547,#40548,#40549,#40550,#40551,#40552,#40553,
#40554,#40555,#40556,#40557,#40558,#40559,#40560,#40561,#40562,#40563,#40564,
#40565,#40566,#40567,#40568,#40569,#40570,#40571,#40572,#40573,#40574,#40575,
#40576,#40577,#40578,#40579,#40580,#40581,#40582,#40583,#40584,#40585,#40586,
#40587,#40588,#40589,#40590,#40591,#40592,#40593,#40594,#40595,#40596,#40597,
#40598,#40599,#40600,#40601,#40602,#40603,#40604,#40605,#40606,#40607,#40608,
#40609,#40610,#40611,#40612,#40613,#40614,#40615,#40616,#40617,#40618,#40619,
#40620,#40621,#40622,#40623,#40624,#40625,#40626,#40627,#40628,#40629,#40630,
#40631,#40632,#40633,#40634,#40635,#40636,#40637,#40638,#40639,#40640,#40641,
#40642,#40643,#40644,#40645,#40646,#40647,#40648,#40649,#40650,#40651,#40652,
#40653,#40654,#40655,#40656,#40657,#40658,#40659,#40660,#40661),
 .UNSPECIFIED.,.F.,.F.,(4,3,3,3,3,3,3,3,3,3,3,3,3,3,3,3,3,3,3,3,3,3,3,3,
3,3,3,3,3,3,3,3,3,3,3,3,3,3,3,3,3,4),(118.464214545145,118.56261566319,
118.66118993359,118.742424380447,118.841022505451,118.939480288228,119.039702856,
119.137982413729,119.236228992802,119.334472075841,119.436169264483,119.534553677901,
119.637907254155,119.741260830409,119.839858955413,119.938316738189,120.038539305962,
120.13681886369,120.235065442764,120.333308525802,120.435005714444,120.533390127863,
120.636743704117,120.740097280371,120.838695405375,120.937153188151,121.037375755924,
121.135655313652,121.233901892726,121.332144975764,121.433842164406,121.532226577825,
121.635580154079,121.738933730333,121.836831200292,121.933909156543,122.030894120917,
122.127817176647,122.226391254986,122.323316910845,122.422715200424,122.522113490002),
 .UNSPECIFIED.);
#316=B_SPLINE_CURVE_WITH_KNOTS('',3,(#40662,#40663,#40664,#40665,#40666,
#40667,#40668),.UNSPECIFIED.,.F.,.F.,(4,1,1,1,4),(122.522113490002,122.737770180294,
123.736606630256,124.735443080218,124.748033420129),.UNSPECIFIED.);
#317=B_SPLINE_CURVE_WITH_KNOTS('',3,(#40670,#40671,#40672,#40673,#40674,
#40675),.UNSPECIFIED.,.F.,.F.,(4,1,1,4),(122.522113490002,123.271799897737,
124.270636347699,124.748072377546),.UNSPECIFIED.);
#318=B_SPLINE_CURVE_WITH_KNOTS('',3,(#40676,#40677,#40678,#40679,#40680,
#40681,#40682,#40683,#40684,#40685,#40686,#40687,#40688,#40689,#40690,#40691,
#40692,#40693,#40694,#40695,#40696,#40697,#40698,#40699,#40700,#40701,#40702,
#40703,#40704,#40705,#40706,#40707,#40708,#40709,#40710,#40711,#40712,#40713,
#40714,#40715,#40716,#40717,#40718,#40719,#40720,#40721,#40722,#40723,#40724,
#40725,#40726,#40727,#40728,#40729,#40730,#40731,#40732,#40733,#40734,#40735,
#40736,#40737,#40738,#40739,#40740,#40741,#40742,#40743,#40744,#40745,#40746,
#40747,#40748,#40749,#40750,#40751,#40752,#40753,#40754,#40755,#40756,#40757,
#40758,#40759,#40760,#40761,#40762,#40763,#40764,#40765,#40766,#40767,#40768,
#40769,#40770,#40771,#40772,#40773,#40774,#40775,#40776,#40777,#40778,#40779,
#40780,#40781,#40782,#40783,#40784,#40785,#40786,#40787,#40788,#40789,#40790,
#40791,#40792,#40793,#40794,#40795,#40796,#40797,#40798,#40799),
 .UNSPECIFIED.,.F.,.F.,(4,3,3,3,3,3,3,3,3,3,3,3,3,3,3,3,3,3,3,3,3,3,3,3,
3,3,3,3,3,3,3,3,3,3,3,3,3,3,3,3,3,4),(118.465360086526,118.566746837947,
118.665030453745,118.763278645539,118.861520898174,118.959786681794,119.058164510988,
119.156609979378,119.255210784522,119.276454097889,119.375052222893,119.47351000567,
119.573732573442,119.67201213117,119.770258710244,119.868501793282,119.970198981925,
120.068583395343,120.171936971597,120.275290547851,120.373888672855,120.472346455631,
120.572569023404,120.670848581132,120.769095160206,120.867338243244,120.969035431886,
121.067419845305,121.170773421559,121.274126997813,121.372725122817,121.471182905593,
121.571405473366,121.669685031094,121.767931610168,121.866174693206,121.967871881848,
122.066256295267,122.169609871521,122.272963447775,122.400857829823,122.522113389964),
 .UNSPECIFIED.);
#319=B_SPLINE_CURVE_WITH_KNOTS('',3,(#40805,#40806,#40807,#40808,#40809,
#40810,#40811,#40812,#40813,#40814,#40815,#40816,#40817,#40818,#40819,#40820,
#40821,#40822,#40823,#40824,#40825,#40826,#40827,#40828,#40829,#40830,#40831,
#40832,#40833,#40834,#40835,#40836,#40837,#40838,#40839,#40840,#40841,#40842,
#40843,#40844,#40845,#40846,#40847,#40848,#40849,#40850,#40851,#40852,#40853,
#40854,#40855,#40856,#40857,#40858,#40859,#40860,#40861,#40862,#40863,#40864,
#40865,#40866,#40867,#40868,#40869,#40870,#40871,#40872,#40873,#40874,#40875,
#40876,#40877,#40878,#40879,#40880,#40881,#40882,#40883,#40884,#40885,#40886,
#40887,#40888,#40889,#40890,#40891,#40892,#40893,#40894,#40895,#40896,#40897,
#40898,#40899,#40900,#40901,#40902,#40903,#40904,#40905,#40906,#40907,#40908,
#40909,#40910,#40911,#40912,#40913,#40914,#40915,#40916,#40917,#40918,#40919,
#40920,#40921,#40922,#40923,#40924,#40925,#40926,#40927,#40928),
 .UNSPECIFIED.,.F.,.F.,(4,3,3,3,3,3,3,3,3,3,3,3,3,3,3,3,3,3,3,3,3,3,3,3,
3,3,3,3,3,3,3,3,3,3,3,3,3,3,3,3,3,4),(112.18179086962,112.280032772378,
112.378281876154,112.47663365233,112.575038389947,112.673614569146,112.749405680676,
112.84800380568,112.946461588456,113.046684156229,113.144963713957,113.243210293031,
113.341453376069,113.443150564711,113.54153497813,113.644888554384,113.748242130638,
113.846840255642,113.945298038418,114.045520606191,114.143800163919,114.242046742992,
114.34028982603,114.441987014672,114.540371428091,114.643725004345,114.747078580599,
114.845676705603,114.94413448838,115.044357056152,115.14263661388,115.240883192953,
115.339126275992,115.440823464634,115.539207878053,115.642561454307,115.745915030561,
115.84988875933,115.953561696348,116.057054365164,116.160309146371,116.238928182547),
 .UNSPECIFIED.);
#320=B_SPLINE_CURVE_WITH_KNOTS('',3,(#40929,#40930,#40931,#40932,#40933,
#40934,#40935,#40936,#40937,#40938,#40939,#40940,#40941,#40942,#40943,#40944,
#40945,#40946,#40947,#40948,#40949,#40950,#40951,#40952,#40953,#40954,#40955,
#40956,#40957,#40958,#40959,#40960,#40961,#40962,#40963,#40964,#40965,#40966,
#40967,#40968,#40969,#40970,#40971,#40972,#40973,#40974,#40975,#40976,#40977,
#40978,#40979,#40980,#40981,#40982,#40983,#40984,#40985,#40986,#40987,#40988,
#40989,#40990,#40991,#40992,#40993,#40994,#40995,#40996,#40997,#40998),
 .UNSPECIFIED.,.F.,.F.,(4,3,3,3,3,3,3,3,3,3,3,3,3,3,3,3,3,3,3,3,3,3,3,4),
(116.238928182823,116.341566510357,116.44447107289,116.547509821617,116.650828963887,
116.744751480523,116.843349605527,116.941807388304,117.042029956076,117.140309513804,
117.238556092878,117.336799175916,117.438496364558,117.536880777977,117.640234354231,
117.743587930485,117.842162082222,117.940606624247,118.03895126967,118.137225626964,
118.235476585645,118.333714612371,118.431998836496,118.464214545145),
 .UNSPECIFIED.);
#321=B_SPLINE_CURVE_WITH_KNOTS('',3,(#41000,#41001,#41002,#41003,#41004,
#41005,#41006,#41007,#41008,#41009,#41010,#41011,#41012,#41013,#41014,#41015,
#41016,#41017,#41018,#41019,#41020,#41021,#41022,#41023,#41024,#41025,#41026,
#41027,#41028,#41029,#41030,#41031,#41032,#41033,#41034,#41035,#41036,#41037,
#41038,#41039,#41040,#41041,#41042,#41043,#41044,#41045,#41046,#41047,#41048,
#41049,#41050,#41051,#41052,#41053,#41054,#41055,#41056,#41057,#41058,#41059,
#41060,#41061,#41062,#41063,#41064,#41065,#41066,#41067,#41068,#41069),
 .UNSPECIFIED.,.F.,.F.,(4,3,3,3,3,3,3,3,3,3,3,3,3,3,3,3,3,3,3,3,3,3,3,4),
(116.238928182823,116.279944748004,116.378542873008,116.477000655784,116.577223223557,
116.675502781285,116.773749360358,116.871992443397,116.973689632039,117.072074045458,
117.175427621712,117.278781197966,117.37737932297,117.475837105746,117.576059673519,
117.674339231247,117.77258581032,117.870828893359,117.972526082001,118.07091049542,
118.174264071673,118.277617647927,118.376189313854,118.465360086526),
 .UNSPECIFIED.);
#322=B_SPLINE_CURVE_WITH_KNOTS('',3,(#41070,#41071,#41072,#41073,#41074,
#41075,#41076,#41077),.UNSPECIFIED.,.F.,.F.,(4,1,1,1,1,4),(112.180986264767,
112.284598948156,113.283435398118,114.28227184808,115.281108298042,116.238922797563),
 .UNSPECIFIED.);
#323=B_SPLINE_CURVE_WITH_KNOTS('',3,(#41083,#41084,#41085,#41086,#41087,
#41088,#41089,#41090,#41091,#41092,#41093,#41094,#41095,#41096,#41097,#41098,
#41099,#41100,#41101,#41102,#41103,#41104,#41105,#41106,#41107,#41108,#41109,
#41110,#41111,#41112,#41113,#41114,#41115,#41116,#41117,#41118,#41119,#41120,
#41121,#41122,#41123,#41124,#41125,#41126,#41127,#41128,#41129,#41130,#41131,
#41132,#41133,#41134,#41135,#41136,#41137,#41138,#41139,#41140,#41141,#41142,
#41143,#41144,#41145,#41146,#41147,#41148,#41149,#41150,#41151,#41152,#41153,
#41154,#41155,#41156,#41157,#41158,#41159,#41160,#41161,#41162,#41163,#41164,
#41165,#41166,#41167,#41168,#41169,#41170,#41171,#41172,#41173,#41174,#41175,
#41176,#41177,#41178,#41179,#41180,#41181,#41182,#41183,#41184,#41185,#41186,
#41187,#41188,#41189,#41190,#41191,#41192,#41193,#41194,#41195,#41196,#41197,
#41198,#41199,#41200,#41201,#41202,#41203,#41204,#41205,#41206),
 .UNSPECIFIED.,.F.,.F.,(4,3,3,3,3,3,3,3,3,3,3,3,3,3,3,3,3,3,3,3,3,3,3,3,
3,3,3,3,3,3,3,3,3,3,3,3,3,3,3,3,3,4),(105.898938865661,105.997345912726,
106.095658421174,106.1939206985,106.292162246928,106.39041254066,106.488766432876,
106.587174674105,106.685752753546,106.756386980904,106.854985105908,106.953442888684,
107.053665456457,107.151945014185,107.250191593259,107.348434676297,107.450131864939,
107.548516278358,107.651869854612,107.755223430866,107.85382155587,107.952279338646,
108.052501906419,108.150781464147,108.249028043221,108.347271126259,108.448968314901,
108.54735272832,108.650706304574,108.754059880828,108.852658005832,108.951115788608,
109.051338356381,109.149617914109,109.247864493183,109.346107576221,109.447804764863,
109.546189178282,109.649542754536,109.75289633079,109.893212936353,109.955742875643),
 .UNSPECIFIED.);
#324=B_SPLINE_CURVE_WITH_KNOTS('',3,(#41207,#41208,#41209,#41210,#41211,
#41212,#41213,#41214,#41215,#41216,#41217,#41218,#41219,#41220,#41221,#41222,
#41223,#41224,#41225,#41226,#41227,#41228,#41229,#41230,#41231,#41232,#41233,
#41234,#41235,#41236,#41237,#41238,#41239,#41240,#41241,#41242,#41243,#41244,
#41245,#41246,#41247,#41248,#41249,#41250,#41251,#41252,#41253,#41254,#41255,
#41256,#41257,#41258,#41259,#41260,#41261,#41262,#41263,#41264,#41265,#41266,
#41267,#41268,#41269,#41270,#41271,#41272,#41273,#41274,#41275,#41276,#41277,
#41278,#41279),.UNSPECIFIED.,.F.,.F.,(4,3,3,3,3,3,3,3,3,3,3,3,3,3,3,3,3,
3,3,3,3,3,3,3,4),(109.955742875951,110.055241614051,110.152151423466,110.249014842069,
110.345862894414,110.447330365999,110.544300028994,110.641334438529,110.738518045248,
110.751732780752,110.850330905756,110.948788688532,111.049011256305,111.147290814033,
111.245537393106,111.343780476145,111.445477664787,111.543862078206,111.64721565446,
111.750569230714,111.849176820424,111.947618966301,112.045965736429,112.144240689708,
112.18179086962),.UNSPECIFIED.);
#325=B_SPLINE_CURVE_WITH_KNOTS('',3,(#41281,#41282,#41283,#41284,#41285,
#41286),.UNSPECIFIED.,.F.,.F.,(4,1,1,4),(109.95575001023,110.286926048232,
111.285762498194,112.180986264767),.UNSPECIFIED.);
#326=B_SPLINE_CURVE_WITH_KNOTS('',3,(#41287,#41288,#41289,#41290,#41291,
#41292,#41293,#41294,#41295,#41296,#41297,#41298,#41299,#41300,#41301,#41302,
#41303,#41304,#41305,#41306,#41307,#41308,#41309,#41310,#41311,#41312,#41313,
#41314,#41315,#41316,#41317,#41318,#41319,#41320,#41321,#41322,#41323,#41324,
#41325,#41326,#41327,#41328,#41329,#41330,#41331,#41332,#41333,#41334,#41335,
#41336,#41337,#41338,#41339,#41340,#41341,#41342,#41343,#41344,#41345,#41346,
#41347,#41348,#41349,#41350,#41351,#41352,#41353,#41354,#41355,#41356,#41357,
#41358,#41359,#41360,#41361,#41362,#41363,#41364,#41365,#41366,#41367,#41368,
#41369,#41370,#41371,#41372,#41373,#41374,#41375,#41376,#41377,#41378,#41379,
#41380,#41381,#41382,#41383,#41384,#41385,#41386,#41387,#41388,#41389,#41390,
#41391,#41392,#41393,#41394,#41395,#41396,#41397,#41398,#41399,#41400,#41401,
#41402,#41403,#41404,#41405,#41406,#41407,#41408,#41409,#41410),
 .UNSPECIFIED.,.F.,.F.,(4,3,3,3,3,3,3,3,3,3,3,3,3,3,3,3,3,3,3,3,3,3,3,3,
3,3,3,3,3,3,3,3,3,3,3,3,3,3,3,3,3,4),(105.898082482581,105.996456924032,
106.09484730115,106.193416271827,106.291580248385,106.390178373389,106.488636156165,
106.588858723938,106.687138281666,106.78538486074,106.883627943778,106.98532513242,
107.083709545839,107.187063122093,107.290416698347,107.389014823351,107.487472606127,
107.5876951739,107.685974731628,107.784221310702,107.88246439374,107.984161582382,
108.082545995801,108.185899572055,108.289253148309,108.387851273313,108.486309056089,
108.586531623862,108.68481118159,108.783057760664,108.881300843702,108.982998032344,
109.081382445763,109.184736022017,109.288089598271,109.386591328536,109.484956309733,
109.583214317042,109.681399820025,109.779540599734,109.877698313766,109.955742875643),
 .UNSPECIFIED.);
#327=B_SPLINE_CURVE_WITH_KNOTS('',3,(#41416,#41417,#41418,#41419,#41420,
#41421,#41422,#41423),.UNSPECIFIED.,.F.,.F.,(4,1,1,1,1,4),(99.6144331696528,
99.7645318311714,100.763368281133,101.762204731095,102.761041181057,103.67254885852),
 .UNSPECIFIED.);
#328=B_SPLINE_CURVE_WITH_KNOTS('',3,(#41424,#41425,#41426,#41427,#41428,
#41429,#41430,#41431,#41432,#41433,#41434,#41435,#41436,#41437,#41438,#41439,
#41440,#41441,#41442,#41443,#41444,#41445,#41446,#41447,#41448,#41449,#41450,
#41451,#41452,#41453,#41454,#41455,#41456,#41457,#41458,#41459,#41460,#41461,
#41462,#41463,#41464,#41465,#41466,#41467,#41468,#41469,#41470,#41471,#41472,
#41473,#41474,#41475,#41476,#41477,#41478,#41479,#41480,#41481,#41482,#41483,
#41484,#41485,#41486,#41487,#41488,#41489,#41490,#41491,#41492,#41493),
 .UNSPECIFIED.,.F.,.F.,(4,3,3,3,3,3,3,3,3,3,3,3,3,3,3,3,3,3,3,3,3,3,3,4),
(103.672557568463,103.759877631019,103.858475756023,103.956933538799,104.057156106572,
104.1554356643,104.253682243374,104.351925326412,104.453622515054,104.552006928473,
104.655360504727,104.758714080981,104.857312205985,104.955769988761,105.055992556534,
105.154272114262,105.252518693335,105.350761776374,105.452458965016,105.550843378435,
105.654196954689,105.757550530943,105.856140410614,105.898938865661),
 .UNSPECIFIED.);
#329=B_SPLINE_CURVE_WITH_KNOTS('',3,(#41495,#41496,#41497,#41498,#41499,
#41500,#41501,#41502,#41503,#41504,#41505,#41506,#41507,#41508,#41509,#41510,
#41511,#41512,#41513,#41514,#41515,#41516,#41517,#41518,#41519,#41520,#41521,
#41522,#41523,#41524,#41525,#41526,#41527,#41528,#41529,#41530,#41531,#41532,
#41533,#41534,#41535,#41536,#41537,#41538,#41539,#41540,#41541,#41542,#41543,
#41544,#41545,#41546,#41547,#41548,#41549,#41550,#41551,#41552,#41553,#41554,
#41555,#41556,#41557,#41558,#41559,#41560,#41561,#41562,#41563,#41564,#41565,
#41566,#41567),.UNSPECIFIED.,.F.,.F.,(4,3,3,3,3,3,3,3,3,3,3,3,3,3,3,3,3,
3,3,3,3,3,3,3,4),(103.672557568463,103.771601702603,103.870660322484,103.96976131202,
104.06899945985,104.168318657834,104.267812431338,104.293907348461,104.392505473465,
104.490963256241,104.591185824014,104.689465381742,104.787711960816,104.885955043854,
104.987652232496,105.086036645915,105.189390222169,105.292743798423,105.391329160737,
105.489781902021,105.591857047161,105.690131953935,105.788367309393,105.88660434371,
105.898082482581),.UNSPECIFIED.);
#330=B_SPLINE_CURVE_WITH_KNOTS('',3,(#41568,#41569,#41570,#41571,#41572,
#41573,#41574,#41575),.UNSPECIFIED.,.F.,.F.,(4,1,1,1,1,4),(99.6160278315589,
100.298561548614,101.297397998576,102.296234448537,103.295070898499,103.672550060583),
 .UNSPECIFIED.);
#331=B_SPLINE_CURVE_WITH_KNOTS('',3,(#41581,#41582,#41583,#41584,#41585,
#41586,#41587,#41588,#41589,#41590,#41591,#41592,#41593,#41594,#41595,#41596,
#41597,#41598,#41599,#41600,#41601,#41602,#41603,#41604,#41605,#41606,#41607,
#41608,#41609,#41610,#41611,#41612,#41613,#41614,#41615,#41616,#41617,#41618,
#41619,#41620,#41621,#41622,#41623,#41624,#41625,#41626,#41627,#41628,#41629,
#41630,#41631,#41632,#41633,#41634,#41635,#41636,#41637,#41638,#41639,#41640,
#41641,#41642,#41643,#41644,#41645,#41646,#41647,#41648,#41649,#41650,#41651,
#41652,#41653,#41654,#41655,#41656,#41657,#41658,#41659,#41660,#41661,#41662,
#41663,#41664,#41665,#41666,#41667,#41668,#41669,#41670,#41671,#41672,#41673,
#41674,#41675,#41676,#41677,#41678,#41679,#41680,#41681,#41682,#41683,#41684,
#41685,#41686,#41687,#41688,#41689,#41690,#41691,#41692,#41693,#41694,#41695,
#41696,#41697,#41698,#41699,#41700,#41701,#41702,#41703,#41704,#41705,#41706,
#41707),.UNSPECIFIED.,.F.,.F.,(4,3,3,3,3,3,3,3,3,3,3,3,3,3,3,3,3,3,3,3,
3,3,3,3,3,3,3,3,3,3,3,3,3,3,3,3,3,3,3,3,3,3,4),(93.3318433927562,93.430100475642,
93.5284654599662,93.6268914127951,93.7254797874492,93.7715131314001,93.8701112564037,
93.9685690391804,94.0687916069531,94.1670711646813,94.2653177437546,94.363560826793,
94.4652580154353,94.5636424288541,94.666996005108,94.770349581362,94.8689477063657,
94.9674054891424,95.067628056915,95.1659076146432,95.2641541937166,95.362397276755,
95.4640944653972,95.562478878816,95.6658324550699,95.7691860313238,95.8677841563276,
95.9662419391042,96.0664645068769,96.1647440646051,96.2629906436785,96.3612337267168,
96.462930915359,96.5613153287778,96.6646689050317,96.7680224812857,96.8674993725788,
96.9668292609828,97.0660403563902,97.1651524247997,97.2642075332236,97.3632407686268,
97.3893722612837),.UNSPECIFIED.);
#332=B_SPLINE_CURVE_WITH_KNOTS('',3,(#41708,#41709,#41710,#41711,#41712,
#41713),.UNSPECIFIED.,.F.,.F.,(4,1,1,4),(97.3893797691262,97.7668589312476,
98.7656953812095,99.6144331696528),.UNSPECIFIED.);
#333=B_SPLINE_CURVE_WITH_KNOTS('',3,(#41715,#41716,#41717,#41718,#41719,
#41720),.UNSPECIFIED.,.F.,.F.,(4,1,1,4),(97.3893809711856,98.3008886486899,
99.2997250986518,99.6160278315589),.UNSPECIFIED.);
#334=B_SPLINE_CURVE_WITH_KNOTS('',3,(#41721,#41722,#41723,#41724,#41725,
#41726,#41727,#41728,#41729,#41730,#41731,#41732,#41733,#41734,#41735,#41736,
#41737,#41738,#41739,#41740,#41741,#41742,#41743,#41744,#41745,#41746,#41747,
#41748,#41749,#41750,#41751,#41752,#41753,#41754,#41755,#41756,#41757,#41758,
#41759,#41760,#41761,#41762,#41763,#41764,#41765,#41766,#41767,#41768,#41769,
#41770,#41771,#41772,#41773,#41774,#41775,#41776,#41777,#41778,#41779,#41780,
#41781,#41782,#41783,#41784,#41785,#41786,#41787,#41788,#41789,#41790,#41791,
#41792,#41793,#41794,#41795,#41796,#41797,#41798,#41799,#41800,#41801,#41802,
#41803,#41804,#41805,#41806,#41807,#41808,#41809,#41810,#41811,#41812,#41813,
#41814,#41815,#41816,#41817,#41818,#41819,#41820,#41821,#41822,#41823,#41824,
#41825,#41826,#41827,#41828,#41829,#41830,#41831,#41832,#41833,#41834,#41835,
#41836,#41837,#41838,#41839,#41840,#41841,#41842,#41843,#41844),
 .UNSPECIFIED.,.F.,.F.,(4,3,3,3,3,3,3,3,3,3,3,3,3,3,3,3,3,3,3,3,3,3,3,3,
3,3,3,3,3,3,3,3,3,3,3,3,3,3,3,3,3,4),(93.3321732640166,93.4307320102719,
93.5291589015738,93.6274833306878,93.7257523216407,93.8239953843585,93.9222419960585,
94.020589057102,94.1189857985572,94.2175578401571,94.3055428488424,94.4041409738461,
94.5025987566228,94.6028213243955,94.7011008821237,94.7993474611971,94.8975905442356,
94.9992877328778,95.0976721462966,95.2010257225504,95.3043792988043,95.402977423808,
95.5014352065847,95.6016577743574,95.6999373320855,95.7981839111589,95.8964269941974,
95.9981241828395,96.0965085962583,96.1998621725122,96.3032157487661,96.4018138737698,
96.5002716565466,96.6004942243192,96.6987737820474,96.7970203611207,96.8952634441592,
96.9969606328014,97.0953450462201,97.1986986224741,97.302052198728,97.3893722612837),
 .UNSPECIFIED.);
#335=B_SPLINE_CURVE_WITH_KNOTS('',3,(#41850,#41851,#41852,#41853,#41854,
#41855,#41856,#41857),.UNSPECIFIED.,.F.,.F.,(4,1,1,1,1,4),(87.0497428708734,
87.7784944316288,88.7773308815907,89.7761673315526,90.7750037815145,91.1061798195662),
 .UNSPECIFIED.);
#336=B_SPLINE_CURVE_WITH_KNOTS('',3,(#41858,#41859,#41860,#41861,#41862,
#41863,#41864,#41865,#41866,#41867,#41868,#41869,#41870,#41871,#41872,#41873,
#41874,#41875,#41876,#41877,#41878,#41879,#41880,#41881,#41882,#41883,#41884,
#41885,#41886,#41887,#41888,#41889,#41890,#41891,#41892,#41893,#41894,#41895,
#41896,#41897,#41898,#41899,#41900,#41901,#41902,#41903,#41904,#41905,#41906,
#41907,#41908,#41909,#41910,#41911,#41912,#41913,#41914,#41915,#41916,#41917,
#41918,#41919,#41920,#41921,#41922,#41923,#41924,#41925,#41926,#41927),
 .UNSPECIFIED.,.F.,.F.,(4,3,3,3,3,3,3,3,3,3,3,3,3,3,3,3,3,3,3,3,3,3,3,4),
(91.1061869541041,91.2043419644769,91.3024795334305,91.4006291648839,91.4988897541855,
91.5972075103077,91.6957053368612,91.7738402314764,91.8724383564801,91.9708961392567,
92.0711187070294,92.1693982647575,92.2676448438309,92.3658879268695,92.4675851155117,
92.5659695289305,92.6693231051843,92.7726766814382,92.8712673172591,92.9697241251359,
93.0680663331458,93.1663410384504,93.2645927043531,93.3318433927562),
 .UNSPECIFIED.);
#337=B_SPLINE_CURVE_WITH_KNOTS('',3,(#41929,#41930,#41931,#41932,#41933,
#41934,#41935,#41936,#41937,#41938,#41939,#41940,#41941,#41942,#41943,#41944,
#41945,#41946,#41947,#41948,#41949,#41950,#41951,#41952,#41953,#41954,#41955,
#41956,#41957,#41958,#41959,#41960,#41961,#41962,#41963,#41964,#41965,#41966,
#41967,#41968,#41969,#41970,#41971,#41972,#41973,#41974,#41975,#41976,#41977,
#41978,#41979,#41980,#41981,#41982,#41983,#41984,#41985,#41986,#41987,#41988,
#41989,#41990,#41991,#41992,#41993,#41994,#41995,#41996,#41997,#41998),
 .UNSPECIFIED.,.F.,.F.,(4,3,3,3,3,3,3,3,3,3,3,3,3,3,3,3,3,3,3,3,3,3,3,4),
(91.1061869541041,91.2465035596787,91.3090334989568,91.4076316239605,91.5060894067373,
91.60631197451,91.7045915322382,91.8028381113116,91.9010811943501,92.0027783829923,
92.1011627964111,92.2045163726649,92.3078699489186,92.4064680739223,92.5049258566991,
92.6051484244717,92.7034279821999,92.8016745612733,92.8999176443118,93.0016148329539,
93.0999992463727,93.2033528226266,93.3067063988805,93.3321732640166),
 .UNSPECIFIED.);
#338=B_SPLINE_CURVE_WITH_KNOTS('',3,(#41999,#42000,#42001,#42002,#42003,
#42004,#42005,#42006,#42007,#42008,#42009,#42010,#42011,#42012,#42013,#42014,
#42015,#42016,#42017,#42018,#42019,#42020,#42021,#42022,#42023,#42024,#42025,
#42026,#42027,#42028,#42029,#42030,#42031,#42032,#42033,#42034,#42035,#42036,
#42037,#42038,#42039,#42040,#42041,#42042,#42043,#42044,#42045,#42046,#42047,
#42048,#42049,#42050,#42051,#42052,#42053,#42054,#42055,#42056,#42057,#42058,
#42059,#42060,#42061,#42062,#42063,#42064,#42065,#42066,#42067,#42068,#42069,
#42070,#42071,#42072,#42073,#42074,#42075,#42076,#42077,#42078,#42079,#42080,
#42081,#42082,#42083,#42084,#42085,#42086,#42087,#42088,#42089,#42090,#42091,
#42092,#42093,#42094,#42095,#42096,#42097,#42098,#42099,#42100,#42101,#42102,
#42103,#42104,#42105,#42106,#42107,#42108,#42109,#42110,#42111,#42112,#42113,
#42114,#42115,#42116,#42117,#42118,#42119,#42120,#42121,#42122,#42123,#42124,
#42125),.UNSPECIFIED.,.F.,.F.,(4,3,3,3,3,3,3,3,3,3,3,3,3,3,3,3,3,3,3,3,
3,3,3,3,3,3,3,3,3,3,3,3,3,3,3,3,3,3,3,3,3,3,4),(87.0482730079683,87.1466827716406,
87.245261692117,87.3136876991093,87.412285824113,87.5107436068897,87.6109661746624,
87.7092457323905,87.8074923114639,87.9057353945024,88.0074325831446,88.1058169965634,
88.2091705728173,88.3125241490712,88.4111222740749,88.5095800568516,88.6098026246243,
88.7080821823525,88.8063287614258,88.9045718444643,89.0062690331065,89.1046534465253,
89.2080070227792,89.311360599033,89.4099587240367,89.5084165068134,89.6086390745861,
89.7069186323142,89.8051652113876,89.9034082944261,90.0051054830683,90.1034898964871,
90.206843472741,90.3101970489949,90.409695787095,90.5067185530535,90.6036495481492,
90.70051989818,90.801936662084,90.8988156754799,90.9957205549589,91.0927209416414,
91.1061869537961),.UNSPECIFIED.);
#339=B_SPLINE_CURVE_WITH_KNOTS('',3,(#42131,#42132,#42133,#42134,#42135,
#42136,#42137,#42138,#42139,#42140,#42141,#42142,#42143,#42144,#42145,#42146,
#42147,#42148,#42149,#42150,#42151,#42152,#42153,#42154,#42155,#42156,#42157,
#42158,#42159,#42160,#42161,#42162,#42163,#42164,#42165,#42166,#42167,#42168,
#42169,#42170,#42171,#42172,#42173,#42174,#42175,#42176,#42177,#42178,#42179,
#42180,#42181,#42182,#42183,#42184,#42185,#42186,#42187,#42188,#42189,#42190,
#42191,#42192,#42193,#42194,#42195,#42196,#42197,#42198,#42199,#42200,#42201,
#42202,#42203,#42204,#42205,#42206,#42207,#42208,#42209,#42210,#42211,#42212,
#42213,#42214,#42215,#42216,#42217,#42218,#42219,#42220,#42221,#42222,#42223,
#42224,#42225,#42226,#42227,#42228,#42229,#42230,#42231,#42232,#42233,#42234,
#42235,#42236,#42237,#42238,#42239,#42240,#42241,#42242,#42243,#42244,#42245,
#42246,#42247,#42248,#42249,#42250,#42251,#42252,#42253,#42254,#42255,#42256,
#42257),.UNSPECIFIED.,.F.,.F.,(4,3,3,3,3,3,3,3,3,3,3,3,3,3,3,3,3,3,3,3,
3,3,3,3,3,3,3,3,3,3,3,3,3,3,3,3,3,3,3,3,3,3,4),(80.765532900003,80.7866392818957,
80.8852374068994,80.9836951896761,81.0839177574488,81.182197315177,81.2804438942504,
81.3786869772888,81.480384165931,81.5787685793498,81.6821221556037,81.7854757318576,
81.8840738568613,81.982531639638,82.0827542074107,82.1810337651389,82.2792803442123,
82.3775234272508,82.479220615893,82.5776050293118,82.6809586055656,82.7843121818195,
82.8829103068232,82.9813680895999,83.0815906573726,83.1798702151008,83.2781167941742,
83.3763598772127,83.4780570658548,83.5764414792737,83.6797950555275,83.7831486317814,
83.8817467567851,83.9802045395619,84.0804271073345,84.1787066650626,84.276953244136,
84.3751963271744,84.4768935158166,84.5752779292354,84.6786315054893,84.7819850817432,
84.8230016469246),.UNSPECIFIED.);
#340=B_SPLINE_CURVE_WITH_KNOTS('',3,(#42258,#42259,#42260,#42261,#42262,
#42263),.UNSPECIFIED.,.F.,.F.,(4,1,1,4),(84.8230070322059,85.7808215317051,
86.779657981667,87.0497428708734),.UNSPECIFIED.);
#341=B_SPLINE_CURVE_WITH_KNOTS('',3,(#42265,#42266,#42267,#42268,#42269,
#42270,#42271,#42272,#42273,#42274,#42275,#42276,#42277,#42278,#42279,#42280,
#42281,#42282,#42283,#42284,#42285,#42286,#42287,#42288,#42289,#42290,#42291,
#42292,#42293,#42294,#42295,#42296,#42297,#42298,#42299,#42300,#42301,#42302,
#42303,#42304,#42305,#42306,#42307,#42308,#42309,#42310,#42311,#42312,#42313,
#42314,#42315,#42316,#42317,#42318,#42319,#42320,#42321,#42322,#42323,#42324,
#42325,#42326,#42327,#42328,#42329,#42330,#42331,#42332,#42333,#42334),
 .UNSPECIFIED.,.F.,.F.,(4,3,3,3,3,3,3,3,3,3,3,3,3,3,3,3,3,3,3,3,3,3,3,4),
(84.8230016472006,84.9261861619504,85.0296647966981,85.1332945907093,85.2372126194225,
85.3160147991855,85.4146129241892,85.513070706966,85.6132932747387,85.7115728324668,
85.8098194115402,85.9080624945788,86.0097596832209,86.1081440966397,86.2114976728936,
86.3148512491474,86.4134243290432,86.5118681332339,86.6102123732759,86.7084866565573,
86.8067399239164,86.9049803913387,87.0032727094089,87.0482730079683),
 .UNSPECIFIED.);
#342=B_SPLINE_CURVE_WITH_KNOTS('',3,(#42335,#42336,#42337,#42338,#42339,
#42340,#42341,#42342,#42343,#42344,#42345,#42346,#42347,#42348,#42349,#42350,
#42351,#42352,#42353,#42354,#42355,#42356,#42357,#42358,#42359,#42360,#42361,
#42362,#42363,#42364,#42365,#42366,#42367,#42368,#42369,#42370,#42371,#42372,
#42373,#42374,#42375,#42376,#42377,#42378,#42379,#42380,#42381,#42382,#42383,
#42384,#42385,#42386,#42387,#42388,#42389,#42390,#42391,#42392,#42393,#42394,
#42395,#42396,#42397,#42398,#42399,#42400,#42401,#42402,#42403,#42404,#42405,
#42406,#42407,#42408,#42409,#42410,#42411,#42412,#42413,#42414,#42415,#42416,
#42417,#42418,#42419,#42420,#42421,#42422,#42423,#42424,#42425,#42426,#42427,
#42428,#42429,#42430,#42431,#42432,#42433,#42434,#42435,#42436,#42437,#42438,
#42439,#42440,#42441,#42442,#42443,#42444,#42445,#42446,#42447,#42448,#42449,
#42450,#42451,#42452,#42453,#42454,#42455,#42456,#42457,#42458),
 .UNSPECIFIED.,.F.,.F.,(4,3,3,3,3,3,3,3,3,3,3,3,3,3,3,3,3,3,3,3,3,3,3,3,
3,3,3,3,3,3,3,3,3,3,3,3,3,3,3,3,3,4),(80.7658264186968,80.8640675910953,
80.9623197955324,81.0606769545392,81.159090517415,81.2576715751211,81.320668999338,
81.4192671243417,81.5177249071185,81.6179474748912,81.7162270326194,81.8144736116928,
81.9127166947314,82.0144138833735,82.1127982967923,82.2161518730461,82.3195054492999,
82.4181035743036,82.5165613570806,82.6167839248532,82.7150634825814,82.8133100616548,
82.9115531446933,83.0132503333354,83.1116347467542,83.214988323008,83.3183418992618,
83.4169400242655,83.5153978070419,83.6156203748147,83.7138999325429,83.8121465116163,
83.9103895946547,84.012086783297,84.1104711967157,84.2138247729697,84.3171783492237,
84.4205578302507,84.5236543867489,84.6265834813182,84.7292989065995,84.8230016469246),
 .UNSPECIFIED.);
#343=B_SPLINE_CURVE_WITH_KNOTS('',3,(#42464,#42465,#42466,#42467,#42468,
#42469,#42470,#42471),.UNSPECIFIED.,.F.,.F.,(4,1,1,1,1,4),(74.4816440654595,
74.7936205821245,75.7924570320864,76.7912934820482,77.7901299320101,78.539816339745),
 .UNSPECIFIED.);
#344=B_SPLINE_CURVE_WITH_KNOTS('',3,(#42472,#42473,#42474,#42475,#42476,
#42477,#42478,#42479,#42480,#42481,#42482,#42483,#42484,#42485,#42486,#42487,
#42488,#42489,#42490,#42491,#42492,#42493,#42494,#42495,#42496,#42497,#42498,
#42499,#42500,#42501,#42502,#42503,#42504,#42505,#42506,#42507,#42508,#42509,
#42510,#42511,#42512,#42513,#42514,#42515,#42516,#42517,#42518,#42519,#42520,
#42521,#42522,#42523,#42524,#42525,#42526,#42527,#42528,#42529,#42530,#42531,
#42532,#42533,#42534,#42535,#42536,#42537,#42538),.UNSPECIFIED.,.F.,.F.,
(4,3,3,3,3,3,3,3,3,3,3,3,3,3,3,3,3,3,3,3,3,3,4),(78.5398164397795,78.6677108218205,
78.788966381972,78.8875645069757,78.9860222897525,79.0862448575251,79.1845244152533,
79.2827709943266,79.3810140773651,79.4827112660073,79.5810956794261,79.68444925568,
79.7878028319339,79.8864023576742,79.984861155696,80.0832042043576,80.1814836418369,
80.279728991266,80.377969735523,80.4762993937422,80.5746716764088,80.6732109326996,
80.765532900003),.UNSPECIFIED.);
#345=B_SPLINE_CURVE_WITH_KNOTS('',3,(#42540,#42541,#42542,#42543,#42544,
#42545,#42546,#42547,#42548,#42549,#42550,#42551,#42552,#42553,#42554,#42555,
#42556,#42557,#42558,#42559,#42560,#42561,#42562,#42563,#42564,#42565,#42566,
#42567,#42568,#42569,#42570,#42571,#42572,#42573,#42574,#42575,#42576,#42577,
#42578,#42579,#42580,#42581,#42582,#42583,#42584,#42585,#42586,#42587,#42588,
#42589,#42590,#42591,#42592,#42593,#42594,#42595,#42596,#42597,#42598,#42599,
#42600,#42601,#42602,#42603,#42604,#42605,#42606,#42607,#42608,#42609),
 .UNSPECIFIED.,.F.,.F.,(4,3,3,3,3,3,3,3,3,3,3,3,3,3,3,3,3,3,3,3,3,3,3,4),
(78.539816339745,78.6377138097037,78.7346673304385,78.8315786913981,78.9284788661295,
79.0271081744507,79.124135318513,79.2235657089636,79.3229960994143,79.421594224418,
79.5200520071949,79.6202745749676,79.7185541326957,79.8168007117691,79.9150437948077,
80.0167409834498,80.1151253968686,80.2184789731224,80.3218325493762,80.4204382921372,
80.5188792313278,80.6172249291511,80.7155010605475,80.7658264186968),
 .UNSPECIFIED.);
#346=B_SPLINE_CURVE_WITH_KNOTS('',3,(#42610,#42611,#42612,#42613,#42614,
#42615,#42616,#42617),.UNSPECIFIED.,.F.,.F.,(4,1,1,1,1,4),(74.4832629992058,
75.3276502995668,76.3264867495287,77.3253231994905,78.3241596494524,78.539816339745),
 .UNSPECIFIED.);
#347=B_SPLINE_CURVE_WITH_KNOTS('',3,(#42623,#42624,#42625,#42626,#42627,
#42628,#42629,#42630,#42631,#42632,#42633,#42634,#42635,#42636,#42637,#42638,
#42639,#42640,#42641,#42642,#42643,#42644,#42645,#42646,#42647,#42648,#42649,
#42650,#42651,#42652,#42653,#42654,#42655,#42656,#42657,#42658,#42659,#42660,
#42661,#42662,#42663,#42664,#42665,#42666,#42667,#42668,#42669,#42670,#42671,
#42672,#42673,#42674,#42675,#42676,#42677,#42678,#42679,#42680,#42681,#42682,
#42683,#42684,#42685,#42686,#42687,#42688,#42689,#42690,#42691,#42692,#42693,
#42694,#42695,#42696,#42697,#42698,#42699,#42700,#42701,#42702,#42703,#42704,
#42705,#42706,#42707,#42708,#42709,#42710,#42711,#42712,#42713,#42714,#42715,
#42716,#42717,#42718,#42719,#42720,#42721,#42722,#42723,#42724,#42725,#42726,
#42727,#42728,#42729,#42730,#42731,#42732,#42733,#42734,#42735,#42736,#42737,
#42738,#42739,#42740,#42741,#42742,#42743,#42744,#42745,#42746),
 .UNSPECIFIED.,.F.,.F.,(4,3,3,3,3,3,3,3,3,3,3,3,3,3,3,3,3,3,3,3,3,3,3,3,
3,3,3,3,3,3,3,3,3,3,3,3,3,3,3,3,3,4),(68.1995885313917,68.2978346979847,
68.3960780479348,68.4972090065394,68.5955944170121,68.6980981496826,68.8006018823532,
68.8992000073569,68.9976577901335,69.0978803579062,69.1961599156344,69.2944064947079,
69.3926495777463,69.4943467663885,69.5927311798074,69.6960847560612,69.7994383323151,
69.8980364573188,69.9964942400958,70.0967168078685,70.1949963655966,70.2932429446698,
70.3914860277081,70.4931832163503,70.5915676297689,70.694921206023,70.798274782277,
70.8968729072807,70.9953306900576,71.0955532578302,71.1938328155585,71.2920793946319,
71.3903224776702,71.4920196663123,71.5904040797312,71.6937576559851,71.7971112322389,
71.9028340905518,72.0081993817381,72.1133399321502,72.2181701837247,72.2566308185864),
 .UNSPECIFIED.);
#348=B_SPLINE_CURVE_WITH_KNOTS('',3,(#42747,#42748,#42749,#42750,#42751,
#42752),.UNSPECIFIED.,.F.,.F.,(4,1,1,4),(72.2566310325654,72.7959476822007,
73.7947841321626,74.4816440654595),.UNSPECIFIED.);
#349=B_SPLINE_CURVE_WITH_KNOTS('',3,(#42754,#42755,#42756,#42757,#42758,
#42759,#42760),.UNSPECIFIED.,.F.,.F.,(4,1,1,1,4),(72.2566310325654,72.3311409496812,
73.329977399643,74.3288138496049,74.4832629992058),.UNSPECIFIED.);
#350=B_SPLINE_CURVE_WITH_KNOTS('',3,(#42761,#42762,#42763,#42764,#42765,
#42766,#42767,#42768,#42769,#42770,#42771,#42772,#42773,#42774,#42775,#42776,
#42777,#42778,#42779,#42780,#42781,#42782,#42783,#42784,#42785,#42786,#42787,
#42788,#42789,#42790,#42791,#42792,#42793,#42794,#42795,#42796,#42797,#42798,
#42799,#42800,#42801,#42802,#42803,#42804,#42805,#42806,#42807,#42808,#42809,
#42810,#42811,#42812,#42813,#42814,#42815,#42816,#42817,#42818,#42819,#42820,
#42821,#42822,#42823,#42824,#42825,#42826,#42827,#42828,#42829,#42830,#42831,
#42832,#42833,#42834,#42835,#42836,#42837,#42838,#42839,#42840,#42841,#42842,
#42843,#42844,#42845,#42846,#42847,#42848,#42849,#42850,#42851,#42852,#42853,
#42854,#42855,#42856,#42857,#42858,#42859,#42860,#42861,#42862,#42863,#42864,
#42865,#42866,#42867,#42868,#42869,#42870,#42871,#42872,#42873,#42874,#42875,
#42876,#42877,#42878,#42879,#42880,#42881,#42882,#42883,#42884,#42885,#42886,
#42887),.UNSPECIFIED.,.F.,.F.,(4,3,3,3,3,3,3,3,3,3,3,3,3,3,3,3,3,3,3,3,
3,3,3,3,3,3,3,3,3,3,3,3,3,3,3,3,3,3,3,3,3,3,4),(68.1987514454805,68.2973434027703,
68.3357951498337,68.4343932748374,68.5328510576141,68.6330736253868,68.7313531831149,
68.8295997621883,68.9278428452268,69.029540033869,69.1279244472877,69.2312780235416,
69.3346315997955,69.4332297247992,69.531687507576,69.6319100753486,69.7301896330768,
69.8284362121502,69.9266792951887,70.0283764838309,70.1267608972497,70.2301144735035,
70.3334680497574,70.4320661747611,70.5305239575379,70.6307465253105,70.7290260830387,
70.8272726621121,70.9255157451506,71.0272129337928,71.1255973472116,71.2289509234654,
71.3323044997193,71.4298807240689,71.5273176349422,71.6246428433671,71.7219081150621,
71.8191441424517,71.9163815796696,72.0137087835221,72.1110862397607,72.2086145464313,
72.2566310325654),.UNSPECIFIED.);
#351=B_SPLINE_CURVE_WITH_KNOTS('',3,(#42893,#42894,#42895,#42896,#42897,
#42898,#42899,#42900),.UNSPECIFIED.,.F.,.F.,(4,1,1,1,1,4),(61.9167164283391,
62.807583182582,63.8064196325439,64.8052560825058,65.8040925324676,65.9734457253857),
 .UNSPECIFIED.);
#352=B_SPLINE_CURVE_WITH_KNOTS('',3,(#42901,#42902,#42903,#42904,#42905,
#42906,#42907,#42908,#42909,#42910,#42911,#42912,#42913,#42914,#42915,#42916,
#42917,#42918,#42919,#42920,#42921,#42922,#42923,#42924,#42925,#42926,#42927,
#42928,#42929,#42930,#42931,#42932,#42933,#42934,#42935,#42936,#42937,#42938,
#42939,#42940,#42941,#42942,#42943,#42944,#42945,#42946,#42947,#42948,#42949,
#42950,#42951,#42952,#42953,#42954,#42955,#42956,#42957,#42958,#42959,#42960,
#42961,#42962,#42963,#42964,#42965,#42966,#42967,#42968,#42969,#42970),
 .UNSPECIFIED.,.F.,.F.,(4,3,3,3,3,3,3,3,3,3,3,3,3,3,3,3,3,3,3,3,3,3,3,4),
(65.9734457253857,66.0704340596178,66.1673127975359,66.2641328887561,66.3609254267911,
66.4577214670339,66.5546134226803,66.6515579893417,66.7486626585401,66.8029289824295,
66.9015271074332,66.9999848902099,67.1002074579826,67.1984870157107,67.2967335947842,
67.3949766778227,67.4966738664649,67.5950582798837,67.6984118561376,67.8017654323914,
67.9012212071415,67.9996662250101,68.0996273782009,68.1995885313917),
 .UNSPECIFIED.);
#353=B_SPLINE_CURVE_WITH_KNOTS('',3,(#42972,#42973,#42974,#42975,#42976,
#42977,#42978,#42979,#42980,#42981,#42982,#42983,#42984,#42985,#42986,#42987,
#42988,#42989,#42990,#42991,#42992,#42993,#42994,#42995,#42996,#42997,#42998,
#42999,#43000,#43001,#43002,#43003,#43004,#43005,#43006,#43007,#43008,#43009,
#43010,#43011,#43012,#43013,#43014,#43015,#43016,#43017,#43018,#43019,#43020,
#43021,#43022,#43023,#43024,#43025,#43026,#43027,#43028,#43029,#43030,#43031,
#43032,#43033,#43034,#43035,#43036,#43037,#43038,#43039,#43040,#43041),
 .UNSPECIFIED.,.F.,.F.,(4,3,3,3,3,3,3,3,3,3,3,3,3,3,3,3,3,3,3,3,3,3,3,4),
(65.9734457256204,66.0848798050745,66.1968635637055,66.3094957826849,66.3381222499099,
66.4367203749136,66.5351781576904,66.635400725463,66.7336802831912,66.8319268622646,
66.9301699453032,67.0318671339454,67.1302515473641,67.233605123618,67.3369586998718,
67.4355663370644,67.5340045943515,67.6323466348136,67.7306220560149,67.8288603843833,
67.9271329658568,68.0254205103276,68.1238183934054,68.1987514454805),
 .UNSPECIFIED.);
#354=B_SPLINE_CURVE_WITH_KNOTS('',3,(#43042,#43043,#43044,#43045,#43046,
#43047,#43048,#43049,#43050,#43051,#43052,#43053,#43054,#43055,#43056,#43057,
#43058,#43059,#43060,#43061,#43062,#43063,#43064,#43065,#43066,#43067,#43068,
#43069,#43070,#43071,#43072,#43073,#43074,#43075,#43076,#43077,#43078,#43079,
#43080,#43081,#43082,#43083,#43084,#43085,#43086,#43087,#43088,#43089,#43090,
#43091,#43092,#43093,#43094,#43095,#43096,#43097,#43098,#43099,#43100,#43101,
#43102,#43103,#43104,#43105,#43106,#43107,#43108,#43109,#43110,#43111,#43112,
#43113,#43114,#43115,#43116,#43117,#43118,#43119,#43120,#43121,#43122,#43123,
#43124,#43125,#43126,#43127,#43128,#43129,#43130,#43131,#43132,#43133,#43134,
#43135,#43136,#43137,#43138,#43139,#43140,#43141,#43142,#43143,#43144,#43145,
#43146,#43147,#43148,#43149,#43150,#43151,#43152,#43153,#43154,#43155,#43156,
#43157,#43158,#43159,#43160,#43161,#43162,#43163,#43164,#43165,#43166,#43167,
#43168),.UNSPECIFIED.,.F.,.F.,(4,3,3,3,3,3,3,3,3,3,3,3,3,3,3,3,3,3,3,3,
3,3,3,3,3,3,3,3,3,3,3,3,3,3,3,3,3,3,3,3,3,3,4),(61.9158792055681,62.0141405477262,
62.1125119549867,62.2109477748074,62.3095423097633,62.3427764500624,62.4413745750661,
62.5398323578432,62.6400549256158,62.738334483344,62.8365810624174,62.9348241454559,
63.036521334098,63.1349057475168,63.2382593237706,63.3416129000243,63.440211025028,
63.538668807805,63.6388913755777,63.7371709333058,63.8354175123792,63.9336605954176,
64.0353577840597,64.1337421974785,64.2370957737324,64.3404493499862,64.4390474749899,
64.5375052577664,64.6377278255391,64.7360073832671,64.8342539623406,64.9324970453788,
65.0341942340211,65.1325786474398,65.2359322236939,65.339285799948,65.4384637976082,
65.5374980774499,65.6364173808601,65.7352455972602,65.8340208922134,65.9327849002204,
65.9734457253857),.UNSPECIFIED.);
#355=B_SPLINE_CURVE_WITH_KNOTS('',3,(#43174,#43175,#43176,#43177,#43178,
#43179,#43180,#43181,#43182,#43183,#43184,#43185,#43186,#43187,#43188,#43189,
#43190,#43191,#43192,#43193,#43194,#43195,#43196,#43197,#43198,#43199,#43200,
#43201,#43202,#43203,#43204,#43205,#43206,#43207,#43208,#43209,#43210,#43211,
#43212,#43213,#43214,#43215,#43216,#43217,#43218,#43219,#43220,#43221,#43222,
#43223,#43224,#43225,#43226,#43227,#43228,#43229,#43230,#43231,#43232,#43233,
#43234,#43235,#43236,#43237,#43238,#43239,#43240,#43241,#43242,#43243,#43244,
#43245,#43246,#43247,#43248,#43249,#43250,#43251,#43252,#43253,#43254,#43255,
#43256,#43257,#43258,#43259,#43260,#43261,#43262,#43263,#43264,#43265,#43266,
#43267,#43268,#43269,#43270,#43271,#43272,#43273,#43274,#43275,#43276,#43277,
#43278,#43279,#43280,#43281,#43282,#43283,#43284,#43285,#43286,#43287,#43288,
#43289,#43290,#43291,#43292,#43293,#43294,#43295,#43296,#43297),
 .UNSPECIFIED.,.F.,.F.,(4,3,3,3,3,3,3,3,3,3,3,3,3,3,3,3,3,3,3,3,3,3,3,3,
3,3,3,3,3,3,3,3,3,3,3,3,3,3,3,3,3,4),(55.6323251401271,55.7308982043818,
55.8157280328489,55.9143261578526,56.0127839406293,56.113006508402,56.2112860661302,
56.3095326452036,56.407775728242,56.5094729168842,56.607857330303,56.7112109065569,
56.8145644828108,56.9131626078145,57.0116203905912,57.1118429583639,57.210122516092,
57.3083690951654,57.4066121782039,57.5083093668461,57.6066937802649,57.7100473565187,
57.8134009327726,57.9119990577762,58.010456840553,58.1106794083257,58.2089589660538,
58.3072055451273,58.4054486281658,58.5071458168079,58.6055302302267,58.7088838064806,
58.8122373827345,58.9094791608007,59.0070768179764,59.1040671063403,59.2009981633324,
59.2979009849175,59.3959908432397,59.4929780422904,59.5916192302483,59.6902604182062),
 .UNSPECIFIED.);
#356=B_SPLINE_CURVE_WITH_KNOTS('',3,(#43298,#43299,#43300,#43301,#43302,
#43303,#43304),.UNSPECIFIED.,.F.,.F.,(4,1,1,1,4),(59.6902604182062,59.8110738326964,
60.8099102826583,61.8087467326201,61.9167164283391),.UNSPECIFIED.);
#357=B_SPLINE_CURVE_WITH_KNOTS('',3,(#43306,#43307,#43308,#43309,#43310,
#43311,#43312,#43313,#43314,#43315,#43316,#43317,#43318,#43319,#43320,#43321,
#43322,#43323,#43324,#43325,#43326,#43327,#43328,#43329,#43330,#43331,#43332,
#43333,#43334,#43335,#43336,#43337,#43338,#43339,#43340,#43341,#43342,#43343,
#43344,#43345,#43346,#43347,#43348,#43349,#43350,#43351,#43352,#43353,#43354,
#43355,#43356,#43357,#43358,#43359,#43360,#43361,#43362,#43363,#43364,#43365,
#43366,#43367,#43368,#43369,#43370,#43371,#43372,#43373,#43374,#43375),
 .UNSPECIFIED.,.F.,.F.,(4,3,3,3,3,3,3,3,3,3,3,3,3,3,3,3,3,3,3,3,3,3,3,4),
(59.6902604182062,59.788634173056,59.8869985815969,59.985382791999,60.0838846667639,
60.1824499292132,60.2811933482969,60.3451035501387,60.4437016751424,60.542159457919,
60.6423820256917,60.7406615834199,60.8389081624932,60.9371512455318,61.038848434174,
61.1372328475928,61.2405864238466,61.3439400001005,61.4425291322825,61.5409847704389,
61.6393272818855,61.7376024228604,61.8358589218425,61.9158792055681),
 .UNSPECIFIED.);
#358=B_SPLINE_CURVE_WITH_KNOTS('',3,(#43376,#43377,#43378,#43379,#43380,
#43381,#43382,#43383,#43384,#43385,#43386,#43387,#43388,#43389,#43390,#43391,
#43392,#43393,#43394,#43395,#43396,#43397,#43398,#43399,#43400,#43401,#43402,
#43403,#43404,#43405,#43406,#43407,#43408,#43409,#43410,#43411,#43412,#43413,
#43414,#43415,#43416,#43417,#43418,#43419,#43420,#43421,#43422,#43423,#43424,
#43425,#43426,#43427,#43428,#43429,#43430,#43431,#43432,#43433,#43434,#43435,
#43436,#43437,#43438,#43439,#43440,#43441,#43442,#43443,#43444,#43445,#43446,
#43447,#43448,#43449,#43450,#43451,#43452,#43453,#43454,#43455,#43456,#43457,
#43458,#43459,#43460,#43461,#43462,#43463,#43464,#43465,#43466,#43467,#43468,
#43469,#43470,#43471,#43472,#43473,#43474,#43475,#43476,#43477,#43478,#43479,
#43480,#43481,#43482,#43483,#43484,#43485,#43486,#43487,#43488,#43489,#43490,
#43491,#43492,#43493,#43494,#43495,#43496,#43497,#43498,#43499),
 .UNSPECIFIED.,.F.,.F.,(4,3,3,3,3,3,3,3,3,3,3,3,3,3,3,3,3,3,3,3,3,3,3,3,
3,3,3,3,3,3,3,3,3,3,3,3,3,3,3,3,3,4),(55.6334624860629,55.7317495305894,
55.8299991741444,55.9282409035089,56.0265041889799,56.124878435732,56.2233185460379,
56.3219158409609,56.3497577502912,56.4483558752949,56.5468136580715,56.6470362258442,
56.7453157835724,56.8435623626458,56.9418054456841,57.0435026343264,57.1418870477452,
57.2452406239991,57.348594200253,57.4471923252568,57.5456501080336,57.6458726758063,
57.7441522335344,57.8423988126078,57.9406418956465,58.0423390842886,58.1407234977073,
58.2440770739611,58.3474306502149,58.4460287752185,58.5444865579953,58.644709125768,
58.7429886834961,58.8412352625696,58.9394783456082,59.0411755342503,59.1395599476692,
59.242913523923,59.3462671001768,59.460882914029,59.5755716660042,59.6902604179793),
 .UNSPECIFIED.);
#359=B_SPLINE_CURVE_WITH_KNOTS('',3,(#43505,#43506,#43507,#43508,#43509,
#43510,#43511,#43512),.UNSPECIFIED.,.F.,.F.,(4,1,1,1,1,4),(49.3495871338273,
49.8227093330776,50.8215457830395,51.8203822330014,52.8192186829633,53.4070751110266),
 .UNSPECIFIED.);
#360=B_SPLINE_CURVE_WITH_KNOTS('',3,(#43513,#43514,#43515,#43516,#43517,
#43518,#43519,#43520,#43521,#43522,#43523,#43524,#43525,#43526,#43527,#43528,
#43529,#43530,#43531,#43532,#43533,#43534,#43535,#43536,#43537,#43538,#43539,
#43540,#43541,#43542,#43543,#43544,#43545,#43546,#43547,#43548,#43549,#43550,
#43551,#43552,#43553,#43554,#43555,#43556,#43557,#43558,#43559,#43560,#43561,
#43562,#43563,#43564,#43565,#43566,#43567,#43568,#43569,#43570,#43571,#43572,
#43573,#43574,#43575,#43576,#43577,#43578,#43579,#43580,#43581,#43582),
 .UNSPECIFIED.,.F.,.F.,(4,3,3,3,3,3,3,3,3,3,3,3,3,3,3,3,3,3,3,3,3,3,3,4),
(53.4070755243489,53.5149520672591,53.6231638610545,53.7318758460054,53.8180551329251,
53.9166532579288,54.0151110407055,54.1153336084782,54.2136131662063,54.3118597452797,
54.4101028283182,54.5118000169604,54.6101844303792,54.7135380066331,54.816891582887,
54.918820777542,55.0172568547355,55.1155965101018,55.2138693416066,55.3121048754619,
55.4103643168845,55.5086391296002,55.6069975818191,55.6323251401271),
 .UNSPECIFIED.);
#361=B_SPLINE_CURVE_WITH_KNOTS('',3,(#43584,#43585,#43586,#43587,#43588,
#43589,#43590,#43591,#43592,#43593,#43594,#43595,#43596,#43597,#43598,#43599,
#43600,#43601,#43602,#43603,#43604,#43605,#43606,#43607,#43608,#43609,#43610,
#43611,#43612,#43613,#43614,#43615,#43616,#43617,#43618,#43619,#43620,#43621,
#43622,#43623,#43624,#43625,#43626,#43627,#43628,#43629,#43630,#43631,#43632,
#43633,#43634,#43635,#43636,#43637,#43638,#43639,#43640,#43641,#43642,#43643,
#43644,#43645,#43646,#43647,#43648,#43649,#43650,#43651,#43652,#43653),
 .UNSPECIFIED.,.F.,.F.,(4,3,3,3,3,3,3,3,3,3,3,3,3,3,3,3,3,3,3,3,3,3,3,4),
(53.4070751110266,53.5048543854907,53.6024983707771,53.7000367768844,53.7975186210124,
53.8949743677961,53.9924344477706,54.0899931990357,54.1876041339867,54.2853815723762,
54.3520848503674,54.4506829753711,54.5491407581481,54.6493633259208,54.7476428836489,
54.8458894627223,54.9441325457608,55.0458297344029,55.1442141478218,55.2475677240755,
55.3509213003293,55.4495112354676,55.5479503969357,55.6334624860629),
 .UNSPECIFIED.);
#362=B_SPLINE_CURVE_WITH_KNOTS('',3,(#43654,#43655,#43656,#43657,#43658,
#43659,#43660,#43661,#43662),.UNSPECIFIED.,.F.,.F.,(4,1,1,1,1,1,4),(49.3496770552549,
49.3579026005581,50.3567390505199,51.3555755004818,52.3544119504437,53.3532484004055,
53.4070751110266),.UNSPECIFIED.);
#363=B_SPLINE_CURVE_WITH_KNOTS('',3,(#43668,#43669,#43670,#43671,#43672,
#43673,#43674,#43675,#43676,#43677,#43678,#43679,#43680,#43681,#43682,#43683,
#43684,#43685,#43686,#43687,#43688,#43689,#43690,#43691,#43692,#43693,#43694,
#43695,#43696,#43697,#43698,#43699,#43700,#43701,#43702,#43703,#43704,#43705,
#43706,#43707,#43708,#43709,#43710,#43711,#43712,#43713,#43714,#43715,#43716,
#43717,#43718,#43719,#43720,#43721,#43722,#43723,#43724,#43725,#43726,#43727,
#43728,#43729,#43730,#43731,#43732,#43733,#43734,#43735,#43736,#43737,#43738,
#43739,#43740,#43741,#43742,#43743,#43744,#43745,#43746,#43747,#43748,#43749,
#43750,#43751,#43752,#43753,#43754,#43755,#43756,#43757,#43758,#43759,#43760,
#43761,#43762,#43763,#43764,#43765,#43766,#43767,#43768,#43769,#43770,#43771,
#43772,#43773,#43774,#43775,#43776,#43777,#43778,#43779,#43780,#43781,#43782,
#43783,#43784,#43785,#43786,#43787,#43788,#43789,#43790,#43791),
 .UNSPECIFIED.,.F.,.F.,(4,3,3,3,3,3,3,3,3,3,3,3,3,3,3,3,3,3,3,3,3,3,3,3,
3,3,3,3,3,3,3,3,3,3,3,3,3,3,3,3,3,4),(43.0671357810666,43.1654506306177,
43.2637141941451,43.3619559753673,43.4602054490314,43.5585578906931,43.6569637353388,
43.7555405095206,43.8296906333064,43.9282887583114,44.0267465410894,44.1269691088618,
44.2252486665913,44.3234952456661,44.4217383287061,44.5234355173466,44.6218199307668,
44.7251735070176,44.8285270832683,44.9271252082716,45.0255829910481,45.1258055588208,
45.2240851165486,45.3223316956214,45.4205747786593,45.522271967302,45.6206563807203,
45.7240099569752,45.8273635332301,45.9259616582337,46.0244194410106,46.1246420087832,
46.2229215665112,46.3211681455844,46.4194112286228,46.5211084172651,46.6194928306838,
46.7228464069379,46.826199983192,46.9466622822371,47.0654828012668,47.1238896269795),
 .UNSPECIFIED.);
#364=B_SPLINE_CURVE_WITH_KNOTS('',3,(#43792,#43793,#43794,#43795,#43796,
#43797),.UNSPECIFIED.,.F.,.F.,(4,1,1,4),(47.123889803847,47.8250364331539,
48.8238728831158,49.3495871338273),.UNSPECIFIED.);
#365=B_SPLINE_CURVE_WITH_KNOTS('',3,(#43799,#43800,#43801,#43802,#43803,
#43804),.UNSPECIFIED.,.F.,.F.,(4,1,1,4),(47.1238901029355,47.3602297006343,
48.3590661505962,49.3496770552549),.UNSPECIFIED.);
#366=B_SPLINE_CURVE_WITH_KNOTS('',3,(#43805,#43806,#43807,#43808,#43809,
#43810,#43811,#43812,#43813,#43814,#43815,#43816,#43817,#43818,#43819,#43820,
#43821,#43822,#43823,#43824,#43825,#43826,#43827,#43828,#43829,#43830,#43831,
#43832,#43833,#43834,#43835,#43836,#43837,#43838,#43839,#43840,#43841,#43842,
#43843,#43844,#43845,#43846,#43847,#43848,#43849,#43850,#43851,#43852,#43853,
#43854,#43855,#43856,#43857,#43858,#43859,#43860,#43861,#43862,#43863,#43864,
#43865,#43866,#43867,#43868,#43869,#43870,#43871,#43872,#43873,#43874,#43875,
#43876,#43877,#43878,#43879,#43880,#43881,#43882,#43883,#43884,#43885,#43886,
#43887,#43888,#43889,#43890,#43891,#43892,#43893,#43894,#43895,#43896,#43897,
#43898,#43899,#43900,#43901,#43902,#43903,#43904,#43905,#43906,#43907,#43908,
#43909,#43910,#43911,#43912,#43913,#43914,#43915,#43916,#43917,#43918,#43919,
#43920,#43921,#43922,#43923,#43924,#43925,#43926,#43927,#43928),
 .UNSPECIFIED.,.F.,.F.,(4,3,3,3,3,3,3,3,3,3,3,3,3,3,3,3,3,3,3,3,3,3,3,3,
3,3,3,3,3,3,3,3,3,3,3,3,3,3,3,3,3,4),(43.0660207258246,43.1644088336187,
43.2646463672028,43.3648839007868,43.4634820258002,43.5619398085867,43.662162376357,
43.7604419340953,43.858688513179,43.9569315962276,44.0586287848579,44.157013198287,
44.2603667745178,44.3637203507487,44.4623184757497,44.5607762585238,44.6609988262972,
44.7592783840227,44.8575249630934,44.9557680461293,45.0574652347747,45.1558496481909,
45.2592032244508,45.3625568007106,45.4611549257133,45.5596127084888,45.6598352762618,
45.7581148339886,45.8563614130607,45.9546044960981,46.0563016847417,46.1546860981592,
46.2580396744158,46.3613932506724,46.4587199838046,46.5559210250952,46.6530274701205,
46.750070296518,46.8471124553622,46.9441490048065,47.0412721236584,47.123889803847),
 .UNSPECIFIED.);
#367=B_SPLINE_CURVE_WITH_KNOTS('',3,(#43934,#43935,#43936,#43937,#43938,
#43939,#43940,#43941,#43942,#43943,#43944,#43945,#43946,#43947,#43948,#43949,
#43950,#43951,#43952,#43953,#43954,#43955,#43956,#43957,#43958,#43959,#43960,
#43961,#43962,#43963,#43964,#43965,#43966,#43967,#43968,#43969,#43970,#43971,
#43972,#43973,#43974,#43975,#43976,#43977,#43978,#43979,#43980,#43981,#43982,
#43983,#43984,#43985,#43986,#43987,#43988,#43989,#43990,#43991,#43992,#43993,
#43994,#43995,#43996,#43997,#43998,#43999,#44000,#44001,#44002,#44003,#44004,
#44005,#44006,#44007,#44008,#44009,#44010,#44011,#44012,#44013,#44014,#44015,
#44016,#44017,#44018,#44019,#44020,#44021,#44022,#44023,#44024,#44025,#44026,
#44027,#44028,#44029,#44030,#44031,#44032,#44033,#44034,#44035,#44036,#44037,
#44038,#44039,#44040,#44041,#44042,#44043,#44044,#44045,#44046,#44047,#44048,
#44049,#44050,#44051,#44052,#44053,#44054,#44055,#44056,#44057,#44058,#44059,
#44060),.UNSPECIFIED.,.F.,.F.,(4,3,3,3,3,3,3,3,3,3,3,3,3,3,3,3,3,3,3,3,
3,3,3,3,3,3,3,3,3,3,3,3,3,3,3,3,3,3,3,3,3,3,4),(36.7830720682974,36.8378354835733,
36.9364336084869,37.0348913911719,37.1351139589673,37.2333935165998,37.3316400955765,
37.4298831785171,37.5315803672716,37.6299647805909,37.7333183570631,37.8366719335352,
37.9352700586074,38.0337278414536,38.1339504092091,38.2322299670085,38.3304765461538,
38.4287196292646,38.5304168178227,38.6288012313141,38.7321548074056,38.835508383497,
38.9341065084865,39.0325642912489,39.1327868590252,39.231066416739,39.3293129957981,
39.4275560788223,39.5292532674815,39.6276376808862,39.7309912571726,39.8343448334589,
39.9329429584521,40.0314007412181,40.1316233089935,40.2299028667105,40.3281494457725,
40.4263925287995,40.5280897174548,40.6264741308619,40.7298277071414,40.8331812834208,
40.8407044966674),.UNSPECIFIED.);
#368=B_SPLINE_CURVE_WITH_KNOTS('',3,(#44061,#44062,#44063,#44064,#44065,
#44066,#44067,#44068,#44069,#44070,#44071,#44072,#44073,#44074,#44075,#44076,
#44077,#44078,#44079,#44080,#44081,#44082,#44083,#44084,#44085,#44086,#44087,
#44088,#44089,#44090,#44091,#44092,#44093,#44094,#44095,#44096,#44097,#44098,
#44099,#44100,#44101,#44102,#44103,#44104,#44105,#44106,#44107,#44108,#44109,
#44110,#44111,#44112,#44113,#44114,#44115,#44116,#44117,#44118,#44119,#44120,
#44121,#44122,#44123,#44124,#44125,#44126,#44127,#44128,#44129,#44130),
 .UNSPECIFIED.,.F.,.F.,(4,3,3,3,3,3,3,3,3,3,3,3,3,3,3,3,3,3,3,3,3,3,3,4),
(40.8407044969197,40.9391705387198,41.037496428004,41.1368115911763,41.2349607512892,
41.3330774110127,41.4311912274061,41.5313978539002,41.6296531901072,41.7308354617449,
41.8320177333826,41.9306158583836,42.0290736411577,42.129296208931,42.2275757666565,
42.3258223457271,42.424065428763,42.5257626174084,42.6241470308245,42.7275006070845,
42.8308541833445,42.9294559188312,43.0279051778647,43.0671357810666),
 .UNSPECIFIED.);
#369=B_SPLINE_CURVE_WITH_KNOTS('',3,(#44132,#44133,#44134,#44135,#44136,
#44137,#44138,#44139,#44140,#44141,#44142,#44143,#44144,#44145,#44146,#44147,
#44148,#44149,#44150,#44151,#44152,#44153,#44154,#44155,#44156,#44157,#44158,
#44159,#44160,#44161,#44162,#44163,#44164,#44165,#44166,#44167,#44168,#44169,
#44170,#44171,#44172,#44173,#44174,#44175,#44176,#44177,#44178,#44179,#44180,
#44181,#44182,#44183,#44184,#44185,#44186,#44187,#44188,#44189,#44190,#44191,
#44192,#44193,#44194,#44195,#44196,#44197,#44198,#44199,#44200,#44201),
 .UNSPECIFIED.,.F.,.F.,(4,3,3,3,3,3,3,3,3,3,3,3,3,3,3,3,3,3,3,3,3,3,3,4),
(40.8407044966674,40.9425310419932,41.0487010317106,41.1508691915795,41.253165848555,
41.355678560324,41.3672110008631,41.4658091258526,41.564266908615,41.6644894763913,
41.7627690341051,41.8610156131641,41.9592586961882,42.0609558848474,42.1593402982522,
42.2626938745385,42.3660474508249,42.4646234053357,42.5630692109104,42.66141458321,
42.7625661188636,42.8608128813695,42.963416803597,43.0660207258246),
 .UNSPECIFIED.);
#370=B_SPLINE_CURVE_WITH_KNOTS('',3,(#44202,#44203,#44204,#44205,#44206,
#44207,#44208,#44209),.UNSPECIFIED.,.F.,.F.,(4,1,1,1,1,4),(36.7838197340187,
37.3718652010156,38.3707016509774,39.3695381009393,40.3683745509012,40.8407024149445),
 .UNSPECIFIED.);
#371=B_SPLINE_CURVE_WITH_KNOTS('',3,(#44215,#44216,#44217,#44218,#44219,
#44220,#44221,#44222,#44223,#44224,#44225,#44226,#44227,#44228,#44229,#44230,
#44231,#44232,#44233,#44234,#44235,#44236,#44237,#44238,#44239,#44240,#44241,
#44242,#44243,#44244,#44245,#44246,#44247,#44248,#44249,#44250,#44251,#44252,
#44253,#44254,#44255,#44256,#44257,#44258,#44259,#44260,#44261,#44262,#44263,
#44264,#44265,#44266,#44267,#44268,#44269,#44270,#44271,#44272,#44273,#44274,
#44275,#44276,#44277,#44278,#44279,#44280,#44281,#44282,#44283,#44284,#44285,
#44286,#44287,#44288,#44289,#44290,#44291,#44292,#44293,#44294,#44295,#44296,
#44297,#44298,#44299,#44300,#44301,#44302,#44303,#44304,#44305,#44306,#44307,
#44308,#44309,#44310,#44311,#44312,#44313,#44314,#44315,#44316,#44317,#44318,
#44319,#44320,#44321,#44322,#44323,#44324,#44325,#44326,#44327,#44328,#44329,
#44330,#44331,#44332,#44333,#44334,#44335,#44336,#44337,#44338,#44339,#44340,
#44341),.UNSPECIFIED.,.F.,.F.,(4,3,3,3,3,3,3,3,3,3,3,3,3,3,3,3,3,3,3,3,
3,3,3,3,3,3,3,3,3,3,3,3,3,3,3,3,3,3,3,3,3,3,4),(30.4997391559443,30.5981023811913,
30.6965255871619,30.7951122973755,30.844816783802,30.9434149029363,31.0418726797402,
31.1420952489931,31.2403748005387,31.3386213733643,31.436864450098,31.5385616460145,
31.6369460530501,31.740299643407,31.8436532337639,31.9422513619608,32.0407091479708,
32.1409317149402,32.2392112759763,32.3374578583783,32.4357009447618,32.5373981295028,
32.6357825462731,32.7391361149995,32.8424896837258,32.9410878085162,33.0395455910849,
33.1397681589102,33.238047716445,33.3362942953307,33.434537378188,33.536234567063,
33.6346189803178,33.7379725570028,33.8413261336877,33.9390973941519,34.0367388270572,
34.1342810926927,34.2317547370095,34.3292101035806,34.4266554953363,34.5241539309141,
34.5575191894878),.UNSPECIFIED.);
#372=B_SPLINE_CURVE_WITH_KNOTS('',3,(#44342,#44343,#44344,#44345,#44346,
#44347,#44348,#44349,#44350,#44351,#44352,#44353,#44354,#44355,#44356,#44357,
#44358,#44359,#44360,#44361,#44362,#44363,#44364,#44365,#44366,#44367,#44368,
#44369,#44370,#44371,#44372,#44373,#44374,#44375,#44376,#44377,#44378,#44379,
#44380,#44381,#44382,#44383,#44384,#44385,#44386,#44387,#44388,#44389,#44390,
#44391,#44392,#44393,#44394,#44395,#44396,#44397,#44398,#44399,#44400,#44401,
#44402,#44403,#44404,#44405,#44406,#44407,#44408,#44409,#44410,#44411),
 .UNSPECIFIED.,.F.,.F.,(4,3,3,3,3,3,3,3,3,3,3,3,3,3,3,3,3,3,3,3,3,3,3,4),
(34.5575191897594,34.6782345503758,34.8009387396348,34.8401625836495,34.9387607091264,
35.0372184923826,35.1374410600362,35.2357206182559,35.3339671978241,35.4322102813602,
35.533907469423,35.6322918833412,35.7356454584763,35.8389990336114,35.9376008413556,
36.0360613066117,36.1344037647116,36.2326817408492,36.3309247589469,36.4291623016086,
36.5274785676935,36.6258371035951,36.7243383499611,36.7830720682974),
 .UNSPECIFIED.);
#373=B_SPLINE_CURVE_WITH_KNOTS('',3,(#44413,#44414,#44415,#44416,#44417,
#44418),.UNSPECIFIED.,.F.,.F.,(4,1,1,4),(34.5575241470784,35.3741923010918,
36.3730287510537,36.7838197340187),.UNSPECIFIED.);
#374=B_SPLINE_CURVE_WITH_KNOTS('',3,(#44419,#44420,#44421,#44422,#44423,
#44424,#44425,#44426,#44427,#44428,#44429,#44430,#44431,#44432,#44433,#44434,
#44435,#44436,#44437,#44438,#44439,#44440,#44441,#44442,#44443,#44444,#44445,
#44446,#44447,#44448,#44449,#44450,#44451,#44452,#44453,#44454,#44455,#44456,
#44457,#44458,#44459,#44460,#44461,#44462,#44463,#44464,#44465,#44466,#44467,
#44468,#44469,#44470,#44471,#44472,#44473,#44474,#44475,#44476,#44477,#44478,
#44479,#44480,#44481,#44482,#44483,#44484,#44485,#44486,#44487,#44488,#44489,
#44490,#44491,#44492,#44493,#44494,#44495,#44496,#44497,#44498,#44499,#44500,
#44501,#44502,#44503,#44504,#44505,#44506,#44507,#44508,#44509,#44510,#44511,
#44512,#44513,#44514,#44515,#44516,#44517,#44518,#44519,#44520,#44521,#44522,
#44523,#44524,#44525,#44526,#44527,#44528,#44529,#44530,#44531,#44532,#44533,
#44534,#44535,#44536,#44537,#44538,#44539,#44540,#44541,#44542),
 .UNSPECIFIED.,.F.,.F.,(4,3,3,3,3,3,3,3,3,3,3,3,3,3,3,3,3,3,3,3,3,3,3,3,
3,3,3,3,3,3,3,3,3,3,3,3,3,3,3,3,3,4),(30.5006743924598,30.599105196373,
30.6974319920214,30.7957023408707,30.8939457544963,30.9921917108564,31.090537495827,
31.188932057399,31.2875029984644,31.3788465012443,31.4774446472446,31.5759024512624,
31.6761250137553,31.7744045931695,31.8726511940475,31.9708942989805,32.0725914620369,
32.1709758973509,32.2743294242786,32.3776829512062,32.4762810765961,32.5747388598255,
32.6749614274933,32.7732409858351,32.8714875655813,32.9697306493509,33.0714278373052,
33.1698122515946,33.2731658263813,33.3765194011681,33.4751175203003,33.5735752971024,
33.6737978663559,33.7720774178991,33.8703239907224,33.9685670674539,34.0702642633729,
34.1686486704062,34.272002260768,34.3753558511299,34.5238559809544,34.5575191894878),
 .UNSPECIFIED.);
#375=B_SPLINE_CURVE_WITH_KNOTS('',3,(#44548,#44549,#44550,#44551,#44552,
#44553,#44554,#44555),.UNSPECIFIED.,.F.,.F.,(4,1,1,1,1,4),(24.2176477571914,
24.8517980840308,25.8506345339927,26.8494709839545,27.8483074339164,28.2743284150372),
 .UNSPECIFIED.);
#376=B_SPLINE_CURVE_WITH_KNOTS('',3,(#44556,#44557,#44558,#44559,#44560,
#44561,#44562,#44563,#44564,#44565,#44566,#44567,#44568,#44569,#44570,#44571,
#44572,#44573,#44574,#44575,#44576,#44577,#44578,#44579,#44580,#44581,#44582,
#44583,#44584,#44585,#44586,#44587,#44588,#44589,#44590,#44591,#44592,#44593,
#44594,#44595,#44596,#44597,#44598,#44599,#44600,#44601,#44602,#44603,#44604,
#44605,#44606,#44607,#44608,#44609,#44610,#44611,#44612,#44613,#44614,#44615,
#44616,#44617,#44618,#44619,#44620,#44621,#44622,#44623,#44624,#44625),
 .UNSPECIFIED.,.F.,.F.,(4,3,3,3,3,3,3,3,3,3,3,3,3,3,3,3,3,3,3,3,3,3,3,4),
(28.2743338823082,28.3746245108422,28.4749734042942,28.5754886326583,28.6760922711292,
28.7769068634701,28.8471438838783,28.9457420298706,29.0441998338806,29.1444223963755,
29.2427019757815,29.3409485766512,29.439191681576,29.540888844642,29.6392732799477,
29.7426268068939,29.8459803338402,29.9445606477316,30.0430096057847,30.1413569295598,
30.2396381186694,30.3378792535517,30.4361386871511,30.4997391559443),
 .UNSPECIFIED.);
#377=B_SPLINE_CURVE_WITH_KNOTS('',3,(#44627,#44628,#44629,#44630,#44631,
#44632,#44633,#44634,#44635,#44636,#44637,#44638,#44639,#44640,#44641,#44642,
#44643,#44644,#44645,#44646,#44647,#44648,#44649,#44650,#44651,#44652,#44653,
#44654,#44655,#44656,#44657,#44658,#44659,#44660,#44661,#44662,#44663,#44664,
#44665,#44666,#44667,#44668,#44669,#44670,#44671,#44672,#44673,#44674,#44675,
#44676,#44677,#44678,#44679,#44680,#44681,#44682,#44683,#44684,#44685,#44686,
#44687,#44688,#44689,#44690,#44691,#44692,#44693,#44694,#44695,#44696),
 .UNSPECIFIED.,.F.,.F.,(4,3,3,3,3,3,3,3,3,3,3,3,3,3,3,3,3,3,3,3,3,3,3,4),
(28.2743338823082,28.3823371513587,28.4809354101241,28.5793933280734,28.6796158622293,
28.7778955576022,28.8761422749412,28.9743854966836,29.0760825228428,29.1744670746393,
29.27782033798,29.3811736013206,29.4797717427214,29.5782295425657,29.6784521061553,
29.7767316824828,29.8749782806886,29.9732213833693,30.0749185503476,30.1733029844888,
30.2766565178856,30.3800100512824,30.4786103666847,30.5006743924598),
 .UNSPECIFIED.);
#378=B_SPLINE_CURVE_WITH_KNOTS('',3,(#44697,#44698,#44699,#44700,#44701,
#44702,#44703,#44704,#44705,#44706,#44707,#44708,#44709,#44710,#44711,#44712,
#44713,#44714,#44715,#44716,#44717,#44718,#44719,#44720,#44721,#44722,#44723,
#44724,#44725,#44726,#44727,#44728,#44729,#44730,#44731,#44732,#44733,#44734,
#44735,#44736,#44737,#44738,#44739,#44740,#44741,#44742,#44743,#44744,#44745,
#44746,#44747,#44748,#44749,#44750,#44751,#44752,#44753,#44754,#44755,#44756,
#44757,#44758,#44759,#44760,#44761,#44762,#44763,#44764,#44765,#44766,#44767,
#44768,#44769,#44770,#44771,#44772,#44773,#44774,#44775,#44776,#44777,#44778,
#44779,#44780,#44781,#44782,#44783,#44784,#44785,#44786,#44787,#44788,#44789,
#44790,#44791,#44792,#44793,#44794,#44795,#44796,#44797,#44798,#44799,#44800,
#44801,#44802,#44803,#44804,#44805,#44806,#44807,#44808,#44809,#44810,#44811,
#44812,#44813,#44814,#44815,#44816,#44817,#44818,#44819,#44820,#44821,#44822,
#44823),.UNSPECIFIED.,.F.,.F.,(4,3,3,3,3,3,3,3,3,3,3,3,3,3,3,3,3,3,3,3,
3,3,3,3,3,3,3,3,3,3,3,3,3,3,3,3,3,3,3,3,3,3,4),(24.2164090613759,24.3149891086871,
24.3869913515112,24.4855869791747,24.584042226434,24.6842654233139,24.7825423701227,
24.8807863158074,24.979026746417,25.080727010181,25.1791087505826,25.2824682760278,
25.3858278014731,25.4844267455965,25.5828853549539,25.683107717014,25.7813881135488,
25.8796355341479,25.9778794603151,26.079575658095,26.1779609099881,26.2813125807115,
26.3846642514349,26.4832625888546,26.5817205901414,26.6819431040484,26.7802228937311,
26.8784697092845,26.9767130330315,27.0784099501228,27.1767946124098,27.2801476569033,
27.3835007013968,27.4808124354761,27.5800026163015,27.6770619119092,27.7740624145151,
27.8710350582304,27.9718597641926,28.0689211628773,28.1660361043295,28.2632831523914,
28.2743338820794),.UNSPECIFIED.);
#379=B_SPLINE_CURVE_WITH_KNOTS('',3,(#44829,#44830,#44831,#44832,#44833,
#44834),.UNSPECIFIED.,.F.,.F.,(4,1,1,4),(15.707963267949,16.3962997518162,
17.3951362017781,17.9335272866486),.UNSPECIFIED.);
#380=B_SPLINE_CURVE_WITH_KNOTS('',3,(#44836,#44837,#44838,#44839,#44840),
 .UNSPECIFIED.,.F.,.F.,(4,1,4),(14.3986268518925,15.3974633018543,15.707963267949),
 .UNSPECIFIED.);
#381=B_SPLINE_CURVE_WITH_KNOTS('',3,(#44844,#44845,#44846,#44847,#44848,
#44849,#44850,#44851,#44852,#44853,#44854,#44855,#44856,#44857,#44858,#44859,
#44860,#44861,#44862,#44863,#44864,#44865,#44866,#44867,#44868,#44869,#44870,
#44871,#44872,#44873,#44874,#44875,#44876,#44877,#44878,#44879,#44880,#44881,
#44882,#44883,#44884,#44885,#44886,#44887,#44888,#44889,#44890,#44891,#44892,
#44893,#44894,#44895,#44896,#44897,#44898,#44899,#44900,#44901),
 .UNSPECIFIED.,.F.,.F.,(4,3,3,3,3,3,3,3,3,3,3,3,3,3,3,3,3,3,3,4),(13.8757070305574,
13.9742332816752,14.0726192270832,14.1714710217493,14.269679438043,14.3678547454402,
14.4660265209369,14.5653782868057,14.6636879754741,14.7635607799431,14.8634335844121,
14.9606976685948,15.0578044132827,15.154822913635,15.2517842191042,15.3487193065272,
15.4457083690103,15.5427241666821,15.6398692546785,15.707963267949),
 .UNSPECIFIED.);
#382=B_SPLINE_CURVE_WITH_KNOTS('',3,(#44902,#44903,#44904,#44905,#44906,
#44907,#44908),.UNSPECIFIED.,.F.,.F.,(4,1,1,1,4),(15.707963267949,15.8622700343739,
16.8611064843358,17.8599429342977,17.9342415312022),.UNSPECIFIED.);
#383=B_SPLINE_CURVE_WITH_KNOTS('',3,(#44914,#44915,#44916,#44917,#44918,
#44919,#44920,#44921),.UNSPECIFIED.,.F.,.F.,(4,1,1,1,1,4),(181.295997131773,
181.669120728045,182.667957178007,183.666793627969,184.665630077931,185.353966561798),
 .UNSPECIFIED.);
#384=B_SPLINE_CURVE_WITH_KNOTS('',3,(#44923,#44924,#44925,#44926,#44927),
 .UNSPECIFIED.,.F.,.F.,(4,1,4),(185.353966561798,185.664466527893,186.663302977854),
 .UNSPECIFIED.);
#385=B_SPLINE_CURVE_WITH_KNOTS('',3,(#44931,#44932,#44933,#44934,#44935,
#44936,#44937,#44938,#44939,#44940,#44941,#44942,#44943,#44944,#44945,#44946,
#44947,#44948,#44949,#44950,#44951,#44952,#44953,#44954,#44955,#44956,#44957,
#44958,#44959,#44960,#44961,#44962,#44963,#44964,#44965,#44966,#44967,#44968,
#44969,#44970,#44971,#44972,#44973,#44974,#44975,#44976,#44977,#44978,#44979,
#44980,#44981,#44982,#44983,#44984,#44985,#44986,#44987,#44988),
 .UNSPECIFIED.,.F.,.F.,(4,3,3,3,3,3,3,3,3,3,3,3,3,3,3,3,3,3,3,4),(185.353966561798,
185.451129857085,185.548173537216,185.645152134409,185.742096640885,185.839038003917,
185.936068669915,186.033145886238,186.130383559937,186.198496245335,186.297011706217,
186.395389165318,186.494243369552,186.592448960961,186.690623574174,186.788796784698,
186.888153288321,186.986469626041,187.086346212615,187.186222799188),
 .UNSPECIFIED.);
#386=B_SPLINE_CURVE_WITH_KNOTS('',3,(#44989,#44990,#44991,#44992,#44993,
#44994,#44995,#44996),.UNSPECIFIED.,.F.,.F.,(4,1,1,1,1,4),(181.297167551772,
182.203150445487,183.201986895449,184.200823345411,185.199659795373,185.353966561798),
 .UNSPECIFIED.);
#387=B_SPLINE_CURVE_WITH_KNOTS('',3,(#45002,#45003,#45004,#45005,#45006,
#45007,#45008,#45009,#45010,#45011,#45012,#45013,#45014,#45015,#45016,#45017,
#45018,#45019,#45020,#45021,#45022,#45023,#45024,#45025,#45026,#45027,#45028,
#45029,#45030,#45031,#45032,#45033,#45034,#45035,#45036,#45037,#45038,#45039,
#45040,#45041,#45042,#45043,#45044,#45045,#45046,#45047,#45048,#45049,#45050,
#45051,#45052,#45053,#45054,#45055,#45056,#45057,#45058,#45059,#45060,#45061,
#45062,#45063,#45064,#45065,#45066,#45067,#45068,#45069,#45070,#45071,#45072,
#45073,#45074,#45075,#45076,#45077,#45078,#45079,#45080,#45081,#45082,#45083,
#45084,#45085,#45086,#45087,#45088,#45089,#45090,#45091,#45092,#45093,#45094,
#45095,#45096,#45097,#45098,#45099,#45100,#45101,#45102,#45103,#45104,#45105,
#45106,#45107,#45108,#45109,#45110,#45111,#45112,#45113,#45114,#45115,#45116,
#45117,#45118,#45119,#45120,#45121,#45122,#45123,#45124,#45125),
 .UNSPECIFIED.,.F.,.F.,(4,3,3,3,3,3,3,3,3,3,3,3,3,3,3,3,3,3,3,3,3,3,3,3,
3,3,3,3,3,3,3,3,3,3,3,3,3,3,3,3,3,4),(175.013888659091,175.112152319873,
175.210394806678,175.308645592818,175.406999705352,175.505407764375,175.603986111103,
175.676102028274,175.774697486027,175.873152598412,175.97337583339,176.071652732112,
176.169896662128,176.268137109468,176.36983745166,176.468219289246,176.571578883741,
176.674938478236,176.773539092151,176.87199934821,176.972221295708,177.070503271274,
177.16875224246,177.266997688919,177.368691998738,177.467078680763,177.570426804481,
177.673774928198,177.772377764237,177.87084030234,177.971061686818,178.069346073265,
178.167597497762,178.265845436446,178.367536921874,178.465926166337,178.569268772248,
178.672611378159,178.782250112465,178.89154546425,179.000249342496,179.070781030154),
 .UNSPECIFIED.);
#388=B_SPLINE_CURVE_WITH_KNOTS('',3,(#45126,#45127,#45128,#45129,#45130,
#45131),.UNSPECIFIED.,.F.,.F.,(4,1,1,4),(179.070781254618,179.671447828121,
180.670284278083,181.295997131773),.UNSPECIFIED.);
#389=B_SPLINE_CURVE_WITH_KNOTS('',3,(#45133,#45134,#45135,#45136,#45137,
#45138,#45139),.UNSPECIFIED.,.F.,.F.,(4,1,1,1,4),(179.070781254618,179.206641095602,
180.205477545564,181.204313995525,181.297167551772),.UNSPECIFIED.);
#390=B_SPLINE_CURVE_WITH_KNOTS('',3,(#45140,#45141,#45142,#45143,#45144,
#45145,#45146,#45147),.UNSPECIFIED.,.F.,.F.,(4,1,1,1,1,4),(175.012544819822,
175.211295295754,176.210131745716,177.208968195678,178.20780464564,179.070781254618),
 .UNSPECIFIED.);
#391=B_SPLINE_CURVE_WITH_KNOTS('',3,(#45153,#45154,#45155,#45156,#45157,
#45158,#45159,#45160,#45161,#45162,#45163,#45164,#45165,#45166,#45167,#45168,
#45169,#45170,#45171,#45172,#45173,#45174,#45175,#45176,#45177,#45178,#45179,
#45180,#45181,#45182,#45183,#45184,#45185,#45186,#45187,#45188,#45189,#45190,
#45191,#45192,#45193,#45194,#45195,#45196,#45197,#45198,#45199,#45200,#45201,
#45202,#45203,#45204,#45205,#45206,#45207,#45208,#45209,#45210,#45211,#45212,
#45213,#45214,#45215,#45216,#45217,#45218,#45219,#45220,#45221,#45222,#45223,
#45224,#45225,#45226,#45227,#45228,#45229,#45230,#45231,#45232,#45233,#45234,
#45235,#45236,#45237,#45238,#45239,#45240,#45241,#45242,#45243,#45244,#45245,
#45246,#45247,#45248,#45249,#45250,#45251,#45252,#45253,#45254,#45255,#45256,
#45257,#45258,#45259,#45260,#45261,#45262,#45263,#45264,#45265,#45266,#45267,
#45268,#45269,#45270,#45271,#45272,#45273,#45274,#45275,#45276),
 .UNSPECIFIED.,.F.,.F.,(4,3,3,3,3,3,3,3,3,3,3,3,3,3,3,3,3,3,3,3,3,3,3,3,
3,3,3,3,3,3,3,3,3,3,3,3,3,3,3,3,3,4),(168.730499547626,168.829027790516,
168.927431100484,169.0257414087,169.124002503139,169.22224388459,169.320495026735,
169.41885037157,169.517260977773,169.615840376683,169.683083328503,169.781681404545,
169.880139138367,169.980361718379,170.078641227516,170.176887758238,170.275130793226,
170.376828039535,170.475212406137,170.578566092301,170.681919778464,170.780517924865,
170.87897572865,170.979198291122,171.077477868766,171.175724467309,171.273967569347,
171.375664734117,171.474049165186,171.577402696806,171.680756228426,171.779354490543,
171.877812411222,171.978034944618,172.076314641176,172.174561359122,172.272804580894,
172.374501605268,172.472886155656,172.576239417022,172.679592678388,172.787595947439),
 .UNSPECIFIED.);
#392=B_SPLINE_CURVE_WITH_KNOTS('',3,(#45277,#45278,#45279,#45280,#45281,
#45282,#45283,#45284,#45285,#45286,#45287,#45288,#45289,#45290,#45291,#45292,
#45293,#45294,#45295,#45296,#45297,#45298,#45299,#45300,#45301,#45302,#45303,
#45304,#45305,#45306,#45307,#45308,#45309,#45310,#45311,#45312,#45313,#45314,
#45315,#45316,#45317,#45318,#45319,#45320,#45321,#45322,#45323,#45324,#45325,
#45326,#45327,#45328,#45329,#45330,#45331,#45332,#45333,#45334,#45335,#45336,
#45337,#45338,#45339,#45340,#45341,#45342,#45343,#45344,#45345,#45346,#45347,
#45348,#45349),.UNSPECIFIED.,.F.,.F.,(4,3,3,3,3,3,3,3,3,3,3,3,3,3,3,3,3,
3,3,3,3,3,3,3,4),(172.787595947668,172.884841558621,172.984040004837,173.081071837019,
173.17805926857,173.275033212353,173.375882191352,173.472980624861,173.57014496835,
173.667458405729,173.67842912835,173.777027506528,173.875485539969,173.975708044762,
174.07398784529,174.172234663731,174.270477982414,174.372174881389,174.470559518877,
174.573912548594,174.677265578312,174.775844828369,174.874301068148,174.972645514908,
175.013888659091),.UNSPECIFIED.);
#393=B_SPLINE_CURVE_WITH_KNOTS('',3,(#45351,#45352,#45353,#45354,#45355,
#45356),.UNSPECIFIED.,.F.,.F.,(4,1,1,4),(172.787601414666,173.21362239583,
174.212458845792,175.012544819822),.UNSPECIFIED.);
#394=B_SPLINE_CURVE_WITH_KNOTS('',3,(#45357,#45358,#45359,#45360,#45361,
#45362,#45363,#45364,#45365,#45366,#45367,#45368,#45369,#45370,#45371,#45372,
#45373,#45374,#45375,#45376,#45377,#45378,#45379,#45380,#45381,#45382,#45383,
#45384,#45385,#45386,#45387,#45388,#45389,#45390,#45391,#45392,#45393,#45394,
#45395,#45396,#45397,#45398,#45399,#45400,#45401,#45402,#45403,#45404,#45405,
#45406,#45407,#45408,#45409,#45410,#45411,#45412,#45413,#45414,#45415,#45416,
#45417,#45418,#45419,#45420,#45421,#45422,#45423,#45424,#45425,#45426,#45427,
#45428,#45429,#45430,#45431,#45432,#45433,#45434,#45435,#45436,#45437,#45438,
#45439,#45440,#45441,#45442,#45443,#45444,#45445,#45446,#45447,#45448,#45449,
#45450,#45451,#45452,#45453,#45454,#45455,#45456,#45457,#45458,#45459,#45460,
#45461,#45462,#45463,#45464,#45465,#45466,#45467,#45468,#45469,#45470,#45471,
#45472,#45473,#45474,#45475,#45476,#45477,#45478,#45479,#45480),
 .UNSPECIFIED.,.F.,.F.,(4,3,3,3,3,3,3,3,3,3,3,3,3,3,3,3,3,3,3,3,3,3,3,3,
3,3,3,3,3,3,3,3,3,3,3,3,3,3,3,3,3,4),(168.730215099249,168.828460566731,
168.926805274994,169.025197908315,169.123767944869,169.218276595983,169.31687471461,
169.415332491016,169.515555060382,169.613834611798,169.712081184595,169.8103242614,
169.912021457536,170.010405864893,170.113759455419,170.217113045945,170.315711171923,
170.414168955616,170.514391523152,170.612671081649,170.710917661434,170.809160745127,
170.910857932822,171.009242346749,171.112595921328,171.215949495907,171.314547642559,
171.413005447084,171.513228009432,171.611507588998,171.709754189896,171.807997294716,
171.909694457505,172.008078892377,172.111432419123,172.214785945869,172.31561776535,
172.416285943722,172.516781875652,172.617176498936,172.717484580452,172.787595947439),
 .UNSPECIFIED.);
#395=B_SPLINE_CURVE_WITH_KNOTS('',3,(#45486,#45487,#45488,#45489,#45490,
#45491,#45492,#45493),.UNSPECIFIED.,.F.,.F.,(4,1,1,1,1,4),(162.44614673284,
162.691228178769,163.690064628731,164.688901078693,165.687737528655,166.504405683219),
 .UNSPECIFIED.);
#396=B_SPLINE_CURVE_WITH_KNOTS('',3,(#45494,#45495,#45496,#45497,#45498,
#45499,#45500,#45501,#45502,#45503,#45504,#45505,#45506,#45507,#45508,#45509,
#45510,#45511,#45512,#45513,#45514,#45515,#45516,#45517,#45518,#45519,#45520,
#45521,#45522,#45523,#45524,#45525,#45526,#45527,#45528,#45529,#45530,#45531,
#45532,#45533,#45534,#45535,#45536,#45537,#45538,#45539,#45540,#45541,#45542,
#45543,#45544,#45545,#45546,#45547,#45548,#45549,#45550,#45551,#45552,#45553,
#45554,#45555,#45556,#45557,#45558,#45559,#45560,#45561,#45562,#45563),
 .UNSPECIFIED.,.F.,.F.,(4,3,3,3,3,3,3,3,3,3,3,3,3,3,3,3,3,3,3,3,3,3,3,4),
(166.504410640259,166.652910770224,166.686573978617,166.785172097217,166.883629873595,
166.983852442968,167.082131994357,167.180378567127,167.278621643905,167.380318840074,
167.478703247404,167.582056837991,167.685410428579,167.784008554554,167.882466338243,
167.98268890578,168.080968464273,168.179215044053,168.277458127742,168.379155315442,
168.477539729364,168.580893303952,168.684246878541,168.730499547626),
 .UNSPECIFIED.);
#397=B_SPLINE_CURVE_WITH_KNOTS('',3,(#45565,#45566,#45567,#45568,#45569,
#45570,#45571,#45572,#45573,#45574,#45575,#45576,#45577,#45578,#45579,#45580,
#45581,#45582,#45583,#45584,#45585,#45586,#45587,#45588,#45589,#45590,#45591,
#45592,#45593,#45594,#45595,#45596,#45597,#45598,#45599,#45600,#45601,#45602,
#45603,#45604,#45605,#45606,#45607,#45608,#45609,#45610,#45611,#45612,#45613,
#45614,#45615,#45616,#45617,#45618,#45619,#45620,#45621,#45622,#45623,#45624,
#45625,#45626,#45627,#45628,#45629,#45630,#45631,#45632,#45633,#45634,#45635,
#45636,#45637),.UNSPECIFIED.,.F.,.F.,(4,3,3,3,3,3,3,3,3,3,3,3,3,3,3,3,3,
3,3,3,3,3,3,3,4),(166.504410640259,166.6019131263,166.699371433809,166.796815990361,
166.894277201725,166.991846173229,167.089478292238,167.18726953544,167.220603696059,
167.319201820915,167.417659603535,167.517882171346,167.616161728898,167.714408307788,
167.812651390637,167.914348579483,168.012732992698,168.11608656936,168.219440146021,
168.318036793093,168.421081369632,168.519419920937,168.617691701668,168.715928374066,
168.730215099249),.UNSPECIFIED.);
#398=B_SPLINE_CURVE_WITH_KNOTS('',3,(#45638,#45639,#45640,#45641,#45642,
#45643,#45644,#45645,#45646,#45647,#45648,#45649,#45650,#45651,#45652,#45653,
#45654,#45655,#45656,#45657,#45658,#45659,#45660,#45661,#45662,#45663,#45664,
#45665,#45666,#45667,#45668,#45669,#45670,#45671,#45672,#45673,#45674,#45675,
#45676,#45677,#45678,#45679,#45680,#45681,#45682,#45683,#45684,#45685,#45686,
#45687,#45688,#45689,#45690,#45691,#45692,#45693,#45694,#45695,#45696,#45697,
#45698,#45699,#45700,#45701,#45702,#45703,#45704,#45705,#45706,#45707,#45708,
#45709,#45710,#45711,#45712,#45713,#45714,#45715,#45716,#45717,#45718,#45719,
#45720,#45721,#45722,#45723,#45724,#45725,#45726,#45727,#45728,#45729,#45730,
#45731,#45732,#45733,#45734,#45735,#45736,#45737,#45738,#45739,#45740,#45741,
#45742,#45743,#45744,#45745,#45746,#45747,#45748,#45749,#45750,#45751,#45752,
#45753,#45754,#45755,#45756,#45757,#45758,#45759,#45760,#45761),
 .UNSPECIFIED.,.F.,.F.,(4,3,3,3,3,3,3,3,3,3,3,3,3,3,3,3,3,3,3,3,3,3,3,3,
3,3,3,3,3,3,3,3,3,3,3,3,3,3,3,3,3,4),(162.4476622356,162.545987531945,162.644257026285,
162.742500229115,162.840746617893,162.939093232495,163.037489201385,163.136060859114,
163.225257896212,163.323856021116,163.422313803793,163.522536371591,163.620815929221,
163.719062508197,163.817305591139,163.919002779898,164.017387193223,164.120740769699,
164.224094346174,164.322692471118,164.421150253833,164.521372821621,164.619652379285,
164.717898958294,164.816142041267,164.917839229984,165.016223643337,165.119577219736,
165.222930796135,165.321528921634,165.419986704907,165.520209272556,165.618488830781,
165.71673541035,165.814978493883,165.916675681936,166.01506009584,166.118413670969,
166.221767246097,166.344599874419,166.465474953174,166.504410639987),
 .UNSPECIFIED.);
#399=B_SPLINE_CURVE_WITH_KNOTS('',3,(#45767,#45768,#45769,#45770,#45771,
#45772,#45773,#45774,#45775,#45776,#45777,#45778,#45779,#45780,#45781,#45782,
#45783,#45784,#45785,#45786,#45787,#45788,#45789,#45790,#45791,#45792,#45793,
#45794,#45795,#45796,#45797,#45798,#45799,#45800,#45801,#45802,#45803,#45804,
#45805,#45806,#45807,#45808,#45809,#45810,#45811,#45812,#45813,#45814,#45815,
#45816,#45817,#45818,#45819,#45820,#45821,#45822,#45823,#45824,#45825,#45826,
#45827,#45828,#45829,#45830,#45831,#45832,#45833,#45834,#45835,#45836,#45837,
#45838,#45839,#45840,#45841,#45842,#45843,#45844,#45845,#45846,#45847,#45848,
#45849,#45850,#45851,#45852,#45853,#45854,#45855,#45856,#45857,#45858,#45859,
#45860,#45861,#45862,#45863,#45864,#45865,#45866,#45867,#45868,#45869,#45870,
#45871,#45872,#45873,#45874,#45875,#45876,#45877,#45878,#45879,#45880,#45881,
#45882,#45883,#45884,#45885,#45886,#45887,#45888,#45889,#45890,#45891,#45892,
#45893),.UNSPECIFIED.,.F.,.F.,(4,3,3,3,3,3,3,3,3,3,3,3,3,3,3,3,3,3,3,3,
3,3,3,3,3,3,3,3,3,3,3,3,3,3,3,3,3,3,3,3,3,3,4),(156.163987593936,156.262228638376,
156.36048690025,156.458853693701,156.557282450291,156.655872547545,156.698209478998,
156.796807604012,156.895265386799,156.995487954569,157.093767512308,157.192014091392,
157.29025717444,157.39195436307,157.490338776499,157.59369235273,157.69704592896,
157.795644053952,157.894101836717,157.994324404493,158.092603962209,158.190850541271,
158.289093624298,158.390790812954,158.489175226362,158.592528802642,158.695882378922,
158.794480503912,158.892938286674,158.993160854451,159.091440412165,159.189686991223,
159.287930074248,159.389627262907,159.488011676311,159.591365252598,159.694718828884,
159.797216560019,159.903218753284,160.005303397592,160.107256278837,160.209067828956,
160.22122533308),.UNSPECIFIED.);
#400=B_SPLINE_CURVE_WITH_KNOTS('',3,(#45894,#45895,#45896,#45897,#45898,
#45899),.UNSPECIFIED.,.F.,.F.,(4,1,1,4),(160.221227414876,160.693555278846,
161.692391728808,162.44614673284),.UNSPECIFIED.);
#401=B_SPLINE_CURVE_WITH_KNOTS('',3,(#45901,#45902,#45903,#45904,#45905,
#45906,#45907,#45908,#45909,#45910,#45911,#45912,#45913,#45914,#45915,#45916,
#45917,#45918,#45919,#45920,#45921,#45922,#45923,#45924,#45925,#45926,#45927,
#45928,#45929,#45930,#45931,#45932,#45933,#45934,#45935,#45936,#45937,#45938,
#45939,#45940,#45941,#45942,#45943,#45944,#45945,#45946,#45947,#45948,#45949,
#45950,#45951,#45952,#45953,#45954,#45955,#45956,#45957,#45958,#45959,#45960,
#45961,#45962,#45963,#45964,#45965,#45966,#45967,#45968,#45969,#45970,#45971,
#45972,#45973),.UNSPECIFIED.,.F.,.F.,(4,3,3,3,3,3,3,3,3,3,3,3,3,3,3,3,3,
3,3,3,3,3,3,3,4),(160.22122533308,160.228748546326,160.327346671318,160.425804454083,
160.526027021859,160.624306579575,160.722553158637,160.820796241665,160.92249343032,
161.020877843728,161.124231420008,161.227584996288,161.326183121278,161.424640904041,
161.524863471817,161.623143029531,161.72138960859,161.819632691614,161.921329880273,
162.019714293678,162.123067869964,162.22642144625,162.325027405982,162.42348150006,
162.4476622356),.UNSPECIFIED.);
#402=B_SPLINE_CURVE_WITH_KNOTS('',3,(#45974,#45975,#45976,#45977,#45978,
#45979,#45980,#45981,#45982,#45983,#45984,#45985,#45986,#45987,#45988,#45989,
#45990,#45991,#45992,#45993,#45994,#45995,#45996,#45997,#45998,#45999,#46000,
#46001,#46002,#46003,#46004,#46005,#46006,#46007,#46008,#46009,#46010,#46011,
#46012,#46013,#46014,#46015,#46016,#46017,#46018,#46019,#46020,#46021,#46022,
#46023,#46024,#46025,#46026,#46027,#46028,#46029,#46030,#46031,#46032,#46033,
#46034,#46035,#46036,#46037,#46038,#46039,#46040,#46041,#46042,#46043,#46044,
#46045,#46046,#46047,#46048,#46049,#46050,#46051,#46052,#46053,#46054,#46055,
#46056,#46057,#46058,#46059,#46060,#46061,#46062,#46063,#46064,#46065,#46066,
#46067,#46068,#46069,#46070,#46071,#46072,#46073,#46074,#46075,#46076,#46077,
#46078,#46079,#46080,#46081,#46082,#46083,#46084,#46085,#46086,#46087,#46088,
#46089,#46090,#46091,#46092,#46093,#46094,#46095,#46096,#46097),
 .UNSPECIFIED.,.F.,.F.,(4,3,3,3,3,3,3,3,3,3,3,3,3,3,3,3,3,3,3,3,3,3,3,3,
3,3,3,3,3,3,3,3,3,3,3,3,3,3,3,3,3,4),(156.163531930331,156.233402746479,
156.332000871484,156.430458654262,156.530681222034,156.628960779764,156.727207358839,
156.825450441878,156.927147630519,157.025532043939,157.128885620189,157.23223919644,
157.330837321442,157.429295104218,157.529517671991,157.627797229718,157.72604380879,
157.824286891827,157.925984080471,158.024368493888,158.127722070145,158.231075646402,
158.329673771403,158.428131554177,158.528354121951,158.626633679676,158.724880258747,
158.823123341783,158.924820530428,159.023204943844,159.126558520104,159.229912096364,
159.328378576654,159.426704810661,159.526019875932,159.624169149677,159.722285836342,
159.820399593048,159.920606027993,160.018861091251,160.120043212039,160.221225332828),
 .UNSPECIFIED.);
#403=B_SPLINE_CURVE_WITH_KNOTS('',3,(#46103,#46104,#46105,#46106,#46107,
#46108,#46109,#46110),.UNSPECIFIED.,.F.,.F.,(4,1,1,1,1,4),(149.881541703048,
150.705190779227,151.704027229189,152.702863679151,153.701700129113,153.93803972631),
 .UNSPECIFIED.);
#404=B_SPLINE_CURVE_WITH_KNOTS('',3,(#46111,#46112,#46113,#46114,#46115,
#46116,#46117,#46118,#46119,#46120,#46121,#46122,#46123,#46124,#46125,#46126,
#46127,#46128,#46129,#46130,#46131,#46132,#46133,#46134,#46135,#46136,#46137,
#46138,#46139,#46140,#46141,#46142,#46143,#46144,#46145,#46146,#46147,#46148,
#46149,#46150,#46151,#46152,#46153,#46154,#46155,#46156,#46157,#46158,#46159,
#46160,#46161,#46162,#46163,#46164,#46165,#46166,#46167,#46168,#46169,#46170,
#46171,#46172,#46173,#46174,#46175,#46176,#46177,#46178,#46179,#46180),
 .UNSPECIFIED.,.F.,.F.,(4,3,3,3,3,3,3,3,3,3,3,3,3,3,3,3,3,3,3,3,3,3,3,4),
(153.9380400259,154.035163898234,154.132222574363,154.229246955325,154.326267897773,
154.423381488606,154.520541056366,154.617870832504,154.700536579074,154.799134704076,
154.897592486852,154.997815054625,155.096094612352,155.194341191424,155.292584274461,
155.394281463105,155.492665876522,155.596019452779,155.699373029036,155.79797586222,
155.89641514303,155.9947593991,156.093038592391,156.163987593936),
 .UNSPECIFIED.);
#405=B_SPLINE_CURVE_WITH_KNOTS('',3,(#46182,#46183,#46184,#46185,#46186,
#46187,#46188,#46189,#46190,#46191,#46192,#46193,#46194,#46195,#46196,#46197,
#46198,#46199,#46200,#46201,#46202,#46203,#46204,#46205,#46206,#46207,#46208,
#46209,#46210,#46211,#46212,#46213,#46214,#46215,#46216,#46217,#46218,#46219,
#46220,#46221,#46222,#46223,#46224,#46225,#46226,#46227,#46228,#46229,#46230,
#46231,#46232,#46233,#46234,#46235,#46236,#46237,#46238,#46239,#46240,#46241,
#46242,#46243,#46244,#46245,#46246,#46247,#46248,#46249,#46250,#46251),
 .UNSPECIFIED.,.F.,.F.,(4,3,3,3,3,3,3,3,3,3,3,3,3,3,3,3,3,3,3,3,3,3,3,4),
(153.938040202764,154.056659980231,154.176963650987,154.235729846555,154.334327971559,
154.432785754335,154.533008322108,154.631287879836,154.729534458909,154.827777541948,
154.92947473059,155.027859144009,155.131212720263,155.234566296517,155.33316914801,
155.431630381046,155.529972651697,155.628250049481,155.726492098717,155.824728281929,
155.923038846792,156.021391522281,156.119876942733,156.163531930331),
 .UNSPECIFIED.);
#406=B_SPLINE_CURVE_WITH_KNOTS('',3,(#46252,#46253,#46254,#46255,#46256,
#46257,#46258,#46259),.UNSPECIFIED.,.F.,.F.,(4,1,1,1,1,4),(149.880018494305,
150.240384046707,151.239220496669,152.238056946631,153.236893396593,153.9380400259),
 .UNSPECIFIED.);
#407=B_SPLINE_CURVE_WITH_KNOTS('',3,(#46265,#46266,#46267,#46268,#46269,
#46270,#46271,#46272,#46273,#46274,#46275,#46276,#46277,#46278,#46279,#46280,
#46281,#46282,#46283,#46284,#46285,#46286,#46287,#46288,#46289,#46290,#46291,
#46292,#46293,#46294,#46295,#46296,#46297,#46298,#46299,#46300,#46301,#46302,
#46303,#46304,#46305,#46306,#46307,#46308,#46309,#46310,#46311,#46312,#46313,
#46314,#46315,#46316,#46317,#46318,#46319,#46320,#46321,#46322,#46323,#46324,
#46325,#46326,#46327,#46328,#46329,#46330,#46331,#46332,#46333,#46334,#46335,
#46336,#46337,#46338,#46339,#46340,#46341,#46342,#46343,#46344,#46345,#46346,
#46347,#46348,#46349,#46350,#46351,#46352,#46353,#46354,#46355,#46356,#46357,
#46358,#46359,#46360,#46361,#46362,#46363,#46364,#46365,#46366,#46367,#46368,
#46369,#46370,#46371,#46372,#46373,#46374,#46375,#46376,#46377,#46378,#46379,
#46380,#46381,#46382,#46383,#46384,#46385,#46386,#46387,#46388,#46389,#46390,
#46391),.UNSPECIFIED.,.F.,.F.,(4,3,3,3,3,3,3,3,3,3,3,3,3,3,3,3,3,3,3,3,
3,3,3,3,3,3,3,3,3,3,3,3,3,3,3,3,3,3,3,3,3,3,4),(143.597018510158,143.695621252539,
143.713335629494,143.811933754498,143.910391537275,144.010614105047,144.108893662775,
144.207140241849,144.305383324887,144.40708051353,144.505464926948,144.608818503202,
144.712172079456,144.81077020446,144.909227987236,145.009450555009,145.107730112737,
145.20597669181,145.304219774849,145.405916963491,145.50430137691,145.607654953164,
145.711008529418,145.809606654422,145.908064437198,146.008287004971,146.106566562699,
146.204813141772,146.303056224811,146.404753413453,146.503137826872,146.606491403125,
146.709844979379,146.807643480436,146.905302408374,147.002849316603,147.100335701354,
147.197792033696,147.295248746519,147.392798083501,147.490396206244,147.588155506493,
147.65485471872),.UNSPECIFIED.);
#408=B_SPLINE_CURVE_WITH_KNOTS('',3,(#46392,#46393,#46394,#46395,#46396,
#46397,#46398),.UNSPECIFIED.,.F.,.F.,(4,1,1,1,4),(147.65485471872,147.708681429341,
148.707517879303,149.706354329265,149.881541703048),.UNSPECIFIED.);
#409=B_SPLINE_CURVE_WITH_KNOTS('',3,(#46400,#46401,#46402,#46403,#46404,
#46405),.UNSPECIFIED.,.F.,.F.,(4,1,1,4),(147.65485471872,148.242711146784,
149.241547596745,149.880018494305),.UNSPECIFIED.);
#410=B_SPLINE_CURVE_WITH_KNOTS('',3,(#46406,#46407,#46408,#46409,#46410,
#46411,#46412,#46413,#46414,#46415,#46416,#46417,#46418,#46419,#46420,#46421,
#46422,#46423,#46424,#46425,#46426,#46427,#46428,#46429,#46430,#46431,#46432,
#46433,#46434,#46435,#46436,#46437,#46438,#46439,#46440,#46441,#46442,#46443,
#46444,#46445,#46446,#46447,#46448,#46449,#46450,#46451,#46452,#46453,#46454,
#46455,#46456,#46457,#46458,#46459,#46460,#46461,#46462,#46463,#46464,#46465,
#46466,#46467,#46468,#46469,#46470,#46471,#46472,#46473,#46474,#46475,#46476,
#46477,#46478,#46479,#46480,#46481,#46482,#46483,#46484,#46485,#46486,#46487,
#46488,#46489,#46490,#46491,#46492,#46493,#46494,#46495,#46496,#46497,#46498,
#46499,#46500,#46501,#46502,#46503,#46504,#46505,#46506,#46507,#46508,#46509,
#46510,#46511,#46512,#46513,#46514,#46515,#46516,#46517,#46518,#46519,#46520,
#46521,#46522,#46523,#46524,#46525,#46526,#46527,#46528,#46529),
 .UNSPECIFIED.,.F.,.F.,(4,3,3,3,3,3,3,3,3,3,3,3,3,3,3,3,3,3,3,3,3,3,3,3,
3,3,3,3,3,3,3,3,3,3,3,3,3,3,3,3,3,4),(143.597933923764,143.696192318378,
143.794433373045,143.892686560447,143.991045348678,144.089461529939,144.188044091191,
144.247365346936,144.34596347194,144.444421254716,144.544643822489,144.642923380217,
144.741169959291,144.839413042329,144.941110230972,145.03949464439,145.142848220644,
145.246201796898,145.344799921902,145.443257704678,145.543480272451,145.641759830179,
145.740006409253,145.838249492291,145.939946680933,146.038331094352,146.141684670606,
146.24503824686,146.343636371864,146.442094154641,146.542316722413,146.640596280141,
146.738842859215,146.837085942253,146.938783130896,147.037167544314,147.140521120568,
147.243874696822,147.352569174392,147.460952550046,147.568802109382,147.654854305401),
 .UNSPECIFIED.);
#411=B_SPLINE_CURVE_WITH_KNOTS('',3,(#46535,#46536,#46537,#46538,#46539,
#46540,#46541,#46542,#46543,#46544,#46545,#46546,#46547,#46548,#46549,#46550,
#46551,#46552,#46553,#46554,#46555,#46556,#46557,#46558,#46559,#46560,#46561,
#46562,#46563,#46564,#46565,#46566,#46567,#46568,#46569,#46570,#46571,#46572,
#46573,#46574,#46575,#46576,#46577,#46578,#46579,#46580,#46581,#46582,#46583,
#46584,#46585,#46586,#46587,#46588,#46589,#46590,#46591,#46592,#46593,#46594,
#46595,#46596,#46597,#46598,#46599,#46600,#46601,#46602,#46603,#46604,#46605,
#46606,#46607,#46608,#46609,#46610,#46611,#46612,#46613,#46614,#46615,#46616,
#46617,#46618,#46619,#46620,#46621,#46622,#46623,#46624,#46625,#46626,#46627,
#46628,#46629,#46630,#46631,#46632,#46633,#46634,#46635,#46636,#46637,#46638,
#46639,#46640,#46641,#46642,#46643,#46644,#46645,#46646,#46647,#46648,#46649,
#46650,#46651,#46652,#46653,#46654,#46655,#46656,#46657,#46658),
 .UNSPECIFIED.,.F.,.F.,(4,3,3,3,3,3,3,3,3,3,3,3,3,3,3,3,3,3,3,3,3,3,3,3,
3,3,3,3,3,3,3,3,3,3,3,3,3,3,3,3,3,4),(137.314044095319,137.41561230392,
137.513996943761,137.617156936742,137.720316929723,137.818915054727,137.917372837503,
138.017595405276,138.115874963004,138.214121542077,138.312364625116,138.414061813758,
138.512446227176,138.61579980343,138.719153379684,138.817751504688,138.916209287464,
139.016431855237,139.114711412965,139.212957992039,139.311201075077,139.412898263719,
139.511282677138,139.614636253392,139.717989829646,139.81658795465,139.915045737427,
140.015268305199,140.113547862927,140.211794442001,140.310037525039,140.411734713681,
140.5101191271,140.613472703354,140.716826279608,140.815569227393,140.914173010821,
141.012667061739,141.111081830931,141.209449097702,141.307822396312,141.371669411541),
 .UNSPECIFIED.);
#412=B_SPLINE_CURVE_WITH_KNOTS('',3,(#46659,#46660,#46661,#46662,#46663,
#46664,#46665,#46666,#46667,#46668,#46669,#46670,#46671,#46672,#46673,#46674,
#46675,#46676,#46677,#46678,#46679,#46680,#46681,#46682,#46683,#46684,#46685,
#46686,#46687,#46688,#46689,#46690,#46691,#46692,#46693,#46694,#46695,#46696,
#46697,#46698,#46699,#46700,#46701,#46702,#46703,#46704,#46705,#46706,#46707,
#46708,#46709,#46710,#46711,#46712,#46713,#46714,#46715,#46716,#46717,#46718,
#46719,#46720,#46721,#46722,#46723,#46724,#46725),.UNSPECIFIED.,.F.,.F.,
(4,3,3,3,3,3,3,3,3,3,3,3,3,3,3,3,3,3,3,3,3,3,4),(141.371669411768,141.485016004534,
141.600339367052,141.71566272957,141.814260854574,141.912718637351,142.012941205123,
142.111220762851,142.209467341925,142.307710424963,142.409407613605,142.507792027024,
142.611145603278,142.714499179532,142.813105314795,142.911543009964,143.009885026327,
143.108160960053,143.206400336867,143.304679404128,143.40297364966,143.501391759162,
143.597018510158),.UNSPECIFIED.);
#413=B_SPLINE_CURVE_WITH_KNOTS('',3,(#46727,#46728,#46729,#46730,#46731,
#46732,#46733,#46734,#46735,#46736,#46737,#46738,#46739,#46740,#46741,#46742,
#46743,#46744,#46745,#46746,#46747,#46748,#46749,#46750,#46751,#46752,#46753,
#46754,#46755,#46756,#46757,#46758,#46759,#46760,#46761,#46762,#46763,#46764,
#46765,#46766,#46767,#46768,#46769,#46770,#46771,#46772,#46773,#46774,#46775,
#46776,#46777,#46778,#46779,#46780,#46781,#46782,#46783,#46784,#46785,#46786,
#46787,#46788,#46789,#46790,#46791,#46792,#46793,#46794,#46795,#46796),
 .UNSPECIFIED.,.F.,.F.,(4,3,3,3,3,3,3,3,3,3,3,3,3,3,3,3,3,3,3,3,3,3,3,4),
(141.371669411541,141.468831254161,141.566438903267,141.66339620349,141.760311911022,
141.857216996242,141.955335858935,142.052368429038,142.151030438025,142.249692447012,
142.348290572016,142.446748354792,142.546970922565,142.645250480293,142.743497059367,
142.841740142405,142.943437331047,143.041821744466,143.14517532072,143.248528896974,
143.3471049557,143.445558136373,143.543900701709,143.597933923764),
 .UNSPECIFIED.);
#414=B_SPLINE_CURVE_WITH_KNOTS('',3,(#46797,#46798,#46799,#46800,#46801,
#46802,#46803,#46804),.UNSPECIFIED.,.F.,.F.,(4,1,1,1,1,4),(137.314688076936,
138.254346647165,139.253183097127,140.252019547089,141.25085599705,141.371669411541),
 .UNSPECIFIED.);
#415=B_SPLINE_CURVE_WITH_KNOTS('',3,(#46810,#46811,#46812,#46813,#46814,
#46815,#46816,#46817,#46818,#46819,#46820,#46821,#46822,#46823,#46824,#46825,
#46826,#46827,#46828,#46829,#46830,#46831,#46832,#46833,#46834,#46835,#46836,
#46837,#46838,#46839,#46840,#46841,#46842,#46843,#46844,#46845,#46846,#46847,
#46848,#46849,#46850,#46851,#46852,#46853,#46854,#46855,#46856,#46857,#46858,
#46859,#46860,#46861,#46862,#46863,#46864,#46865,#46866,#46867,#46868,#46869,
#46870,#46871,#46872,#46873,#46874,#46875,#46876,#46877,#46878,#46879,#46880,
#46881,#46882,#46883,#46884,#46885,#46886,#46887,#46888,#46889,#46890,#46891,
#46892,#46893,#46894,#46895,#46896,#46897,#46898,#46899,#46900,#46901,#46902,
#46903,#46904,#46905,#46906,#46907,#46908,#46909,#46910,#46911,#46912,#46913,
#46914,#46915,#46916,#46917,#46918,#46919,#46920,#46921,#46922,#46923,#46924,
#46925,#46926,#46927,#46928,#46929,#46930,#46931,#46932,#46933),
 .UNSPECIFIED.,.F.,.F.,(4,3,3,3,3,3,3,3,3,3,3,3,3,3,3,3,3,3,3,3,3,3,3,3,
3,3,3,3,3,3,3,3,3,3,3,3,3,3,3,3,3,4),(131.031654973638,131.129931712951,
131.228177248346,131.326421060941,131.426640353193,131.525027385579,131.626162807765,
131.727298229951,131.825896354955,131.924354137732,132.024576705504,132.122856263233,
132.221102842306,132.319345925345,132.421043113987,132.519427527405,132.622781103659,
132.726134679913,132.824732804917,132.923190587694,133.023413155466,133.121692713194,
133.219939292268,133.318182375306,133.419879563948,133.518263977367,133.621617553621,
133.724971129875,133.823569254879,133.922027037656,134.022249605428,134.120529163156,
134.21877574223,134.317018825268,134.418716013911,134.517100427329,134.620454003583,
134.723807579837,134.8363385207,134.948409000641,135.059693750754,135.088484104126),
 .UNSPECIFIED.);
#416=B_SPLINE_CURVE_WITH_KNOTS('',3,(#46934,#46935,#46936,#46937,#46938,
#46939,#46940,#46941,#46942,#46943,#46944,#46945,#46946,#46947,#46948,#46949,
#46950,#46951,#46952,#46953,#46954,#46955,#46956,#46957,#46958,#46959,#46960,
#46961,#46962,#46963,#46964,#46965,#46966,#46967,#46968,#46969,#46970,#46971,
#46972,#46973,#46974,#46975,#46976,#46977,#46978,#46979,#46980,#46981,#46982,
#46983,#46984,#46985,#46986,#46987,#46988,#46989,#46990,#46991,#46992,#46993,
#46994,#46995,#46996,#46997,#46998,#46999,#47000,#47001,#47002,#47003),
 .UNSPECIFIED.,.F.,.F.,(4,3,3,3,3,3,3,3,3,3,3,3,3,3,3,3,3,3,3,3,3,3,3,4),
(135.088484104361,135.187254556185,135.286029876604,135.384838499174,135.483776463585,
135.582788468008,135.681976179005,135.722644029799,135.821242154803,135.919699937579,
136.019922505352,136.11820206308,136.216448642154,136.314691725192,136.416388913834,
136.514773327253,136.618126903507,136.721480479761,136.82006725633,136.918521077985,
137.017401832319,137.115677672201,137.21486088376,137.314044095319),
 .UNSPECIFIED.);
#417=B_SPLINE_CURVE_WITH_KNOTS('',3,(#47005,#47006,#47007,#47008,#47009,
#47010,#47011),.UNSPECIFIED.,.F.,.F.,(4,1,1,1,4),(135.088484104361,135.257837297279,
136.256673747241,137.255510197203,137.314688076936),.UNSPECIFIED.);
#418=B_SPLINE_CURVE_WITH_KNOTS('',3,(#47012,#47013,#47014,#47015,#47016,
#47017,#47018,#47019,#47020,#47021,#47022,#47023,#47024,#47025,#47026,#47027,
#47028,#47029,#47030,#47031,#47032,#47033,#47034,#47035,#47036,#47037,#47038,
#47039,#47040,#47041,#47042,#47043,#47044,#47045,#47046,#47047,#47048,#47049,
#47050,#47051,#47052,#47053,#47054,#47055,#47056,#47057,#47058,#47059,#47060,
#47061,#47062,#47063,#47064,#47065,#47066,#47067,#47068,#47069,#47070,#47071,
#47072,#47073,#47074,#47075,#47076,#47077,#47078,#47079,#47080,#47081,#47082,
#47083,#47084,#47085,#47086,#47087,#47088,#47089,#47090,#47091,#47092,#47093,
#47094,#47095,#47096,#47097,#47098,#47099,#47100,#47101,#47102,#47103,#47104,
#47105,#47106,#47107,#47108,#47109,#47110,#47111,#47112,#47113,#47114,#47115,
#47116,#47117,#47118,#47119,#47120,#47121,#47122,#47123,#47124,#47125,#47126,
#47127,#47128,#47129,#47130,#47131,#47132,#47133,#47134,#47135,#47136,#47137,
#47138),.UNSPECIFIED.,.F.,.F.,(4,3,3,3,3,3,3,3,3,3,3,3,3,3,3,3,3,3,3,3,
3,3,3,3,3,3,3,3,3,3,3,3,3,3,3,3,3,3,3,3,3,3,4),(131.030544944991,131.128979440939,
131.227573133845,131.262491497432,131.361089622436,131.459547405212,131.559769972985,
131.658049530713,131.756296109787,131.854539192825,131.956236381467,132.054620794886,
132.15797437114,132.261327947394,132.359926072398,132.458383855174,132.558606422947,
132.656885980675,132.755132559748,132.853375642787,132.955072831429,133.053457244848,
133.156810821101,133.260164397355,133.358762522359,133.457220305135,133.557442872908,
133.655722430636,133.753969009709,133.852212092748,133.95390928139,134.052293694809,
134.155647271063,134.259000847317,134.356128675187,134.453094160804,134.549968416923,
134.6467826177,134.743567858739,134.84039997176,134.937256811787,135.034231214226,
135.088484104361),.UNSPECIFIED.);
#419=B_SPLINE_CURVE_WITH_KNOTS('',3,(#47144,#47145,#47146,#47147,#47148,
#47149,#47150,#47151),.UNSPECIFIED.,.F.,.F.,(4,1,1,1,1,4),(124.748033484277,
125.73427953018,126.733115980142,127.731952430104,128.730788880066,128.805298797182),
 .UNSPECIFIED.);
#420=B_SPLINE_CURVE_WITH_KNOTS('',3,(#47152,#47153,#47154,#47155,#47156,
#47157,#47158,#47159,#47160,#47161,#47162,#47163,#47164,#47165,#47166,#47167,
#47168,#47169,#47170,#47171,#47172,#47173,#47174,#47175,#47176,#47177,#47178,
#47179,#47180,#47181,#47182,#47183,#47184,#47185,#47186,#47187,#47188,#47189,
#47190,#47191,#47192,#47193,#47194,#47195,#47196,#47197,#47198,#47199,#47200,
#47201,#47202,#47203,#47204,#47205,#47206,#47207,#47208,#47209,#47210,#47211,
#47212,#47213,#47214,#47215,#47216,#47217,#47218,#47219,#47220,#47221),
 .UNSPECIFIED.,.F.,.F.,(4,3,3,3,3,3,3,3,3,3,3,3,3,3,3,3,3,3,3,3,3,3,3,4),
(128.805298797182,128.902840431273,129.000250613517,129.097560812666,129.194818343698,
129.292053887498,129.389298094495,129.486642967569,129.584044330746,129.681605924981,
129.729625330028,129.828223455032,129.926681237808,130.026903805581,130.125183363309,
130.223429942382,130.321673025421,130.423370214063,130.521754627482,130.625108203735,
130.728461779989,130.82704702784,130.929351000739,131.031654973638),
 .UNSPECIFIED.);
#421=B_SPLINE_CURVE_WITH_KNOTS('',3,(#47223,#47224,#47225,#47226,#47227,
#47228,#47229,#47230,#47231,#47232,#47233,#47234,#47235,#47236,#47237,#47238,
#47239,#47240,#47241,#47242,#47243,#47244,#47245,#47246,#47247,#47248,#47249,
#47250,#47251,#47252,#47253,#47254,#47255,#47256,#47257,#47258,#47259,#47260,
#47261,#47262,#47263,#47264,#47265,#47266,#47267,#47268,#47269,#47270,#47271,
#47272,#47273,#47274,#47275,#47276,#47277,#47278,#47279,#47280,#47281,#47282,
#47283,#47284,#47285,#47286,#47287,#47288,#47289,#47290,#47291,#47292),
 .UNSPECIFIED.,.F.,.F.,(4,3,3,3,3,3,3,3,3,3,3,3,3,3,3,3,3,3,3,3,3,3,3,4),
(128.805299011159,128.91008561987,129.01525575915,129.120630109632,129.226318351047,
129.264818597508,129.363416722512,129.461874505288,129.562097073061,129.660376630789,
129.758623209863,129.856866292901,129.958563481543,130.056947894962,130.160301471216,
130.26365504747,130.362225486655,130.460667523599,130.55901086589,130.657285118175,
130.755545076206,130.853792579363,130.952108672697,131.030544944991),
 .UNSPECIFIED.);
#422=B_SPLINE_CURVE_WITH_KNOTS('',3,(#47293,#47294,#47295,#47296,#47297,
#47298,#47299,#47300),.UNSPECIFIED.,.F.,.F.,(4,1,1,1,1,4),(124.748072441043,
125.26947279766,126.268309247622,127.267145697584,128.265982147546,128.805298797182),
 .UNSPECIFIED.);
#423=B_SPLINE_CURVE_WITH_KNOTS('',3,(#47306,#47307,#47308,#47309,#47310,
#47311,#47312,#47313,#47314,#47315,#47316,#47317,#47318,#47319,#47320,#47321,
#47322,#47323,#47324,#47325,#47326,#47327,#47328,#47329,#47330,#47331,#47332,
#47333,#47334,#47335,#47336,#47337,#47338,#47339,#47340,#47341,#47342,#47343,
#47344,#47345,#47346,#47347,#47348,#47349,#47350,#47351,#47352,#47353,#47354,
#47355,#47356,#47357,#47358,#47359,#47360,#47361,#47362,#47363,#47364,#47365,
#47366,#47367,#47368,#47369,#47370,#47371,#47372,#47373,#47374,#47375,#47376,
#47377,#47378,#47379,#47380,#47381,#47382,#47383,#47384,#47385,#47386,#47387,
#47388,#47389,#47390,#47391,#47392,#47393,#47394,#47395,#47396,#47397,#47398,
#47399,#47400,#47401,#47402,#47403,#47404,#47405,#47406,#47407,#47408,#47409,
#47410,#47411,#47412,#47413,#47414,#47415,#47416,#47417,#47418,#47419,#47420,
#47421,#47422,#47423,#47424,#47425,#47426,#47427,#47428,#47429),
 .UNSPECIFIED.,.F.,.F.,(4,3,3,3,3,3,3,3,3,3,3,3,3,3,3,3,3,3,3,3,3,3,3,3,
3,3,3,3,3,3,3,3,3,3,3,3,3,3,3,3,3,4),(118.464214608881,118.562615726968,
118.661189997389,118.742424380447,118.841022505451,118.939480288228,119.039702856,
119.137982413728,119.236228992802,119.33447207584,119.436169264482,119.534553677901,
119.637907254155,119.741260830409,119.839858955413,119.93831673819,120.038539305962,
120.136818863691,120.235065442764,120.333308525803,120.435005714445,120.533390127863,
120.636743704117,120.740097280371,120.838695405375,120.937153188151,121.037375755924,
121.135655313652,121.233901892726,121.332144975764,121.433842164406,121.532226577825,
121.635580154079,121.738933730333,121.836831200292,121.933909156543,122.030894120917,
122.127817176647,122.226391254986,122.323316910845,122.422715200423,122.522113490002),
 .UNSPECIFIED.);
#424=B_SPLINE_CURVE_WITH_KNOTS('',3,(#47430,#47431,#47432,#47433,#47434,
#47435,#47436),.UNSPECIFIED.,.F.,.F.,(4,1,1,1,4),(122.522113490002,122.737770180294,
123.736606630256,124.735443080218,124.748033484277),.UNSPECIFIED.);
#425=B_SPLINE_CURVE_WITH_KNOTS('',3,(#47438,#47439,#47440,#47441,#47442,
#47443),.UNSPECIFIED.,.F.,.F.,(4,1,1,4),(122.522113490002,123.271799897737,
124.270636347699,124.748072441043),.UNSPECIFIED.);
#426=B_SPLINE_CURVE_WITH_KNOTS('',3,(#47444,#47445,#47446,#47447,#47448,
#47449,#47450,#47451,#47452,#47453,#47454,#47455,#47456,#47457,#47458,#47459,
#47460,#47461,#47462,#47463,#47464,#47465,#47466,#47467,#47468,#47469,#47470,
#47471,#47472,#47473,#47474,#47475,#47476,#47477,#47478,#47479,#47480,#47481,
#47482,#47483,#47484,#47485,#47486,#47487,#47488,#47489,#47490,#47491,#47492,
#47493,#47494,#47495,#47496,#47497,#47498,#47499,#47500,#47501,#47502,#47503,
#47504,#47505,#47506,#47507,#47508,#47509,#47510,#47511,#47512,#47513,#47514,
#47515,#47516,#47517,#47518,#47519,#47520,#47521,#47522,#47523,#47524,#47525,
#47526,#47527,#47528,#47529,#47530,#47531,#47532,#47533,#47534,#47535,#47536,
#47537,#47538,#47539,#47540,#47541,#47542,#47543,#47544,#47545,#47546,#47547,
#47548,#47549,#47550,#47551,#47552,#47553,#47554,#47555,#47556,#47557,#47558,
#47559,#47560,#47561,#47562,#47563,#47564,#47565,#47566,#47567),
 .UNSPECIFIED.,.F.,.F.,(4,3,3,3,3,3,3,3,3,3,3,3,3,3,3,3,3,3,3,3,3,3,3,3,
3,3,3,3,3,3,3,3,3,3,3,3,3,3,3,3,3,4),(118.465360150378,118.566746893817,
118.665030509587,118.763278701368,118.861520954009,118.959786737651,119.058164566875,
119.156610035311,119.255210840485,119.276454097889,119.375052222893,119.47351000567,
119.573732573442,119.67201213117,119.770258710244,119.868501793282,119.970198981924,
120.068583395343,120.171936971597,120.275290547851,120.373888672855,120.472346455631,
120.572569023404,120.670848581132,120.769095160206,120.867338243244,120.969035431886,
121.067419845305,121.170773421559,121.274126997813,121.372725122817,121.471182905594,
121.571405473366,121.669685031094,121.767931610168,121.866174693206,121.967871881848,
122.066256295267,122.169609871521,122.272963447775,122.40085782982,122.522113389975),
 .UNSPECIFIED.);
#427=B_SPLINE_CURVE_WITH_KNOTS('',3,(#47573,#47574,#47575,#47576,#47577,
#47578,#47579,#47580,#47581,#47582,#47583,#47584,#47585,#47586,#47587,#47588,
#47589,#47590,#47591,#47592,#47593,#47594,#47595,#47596,#47597,#47598,#47599,
#47600,#47601,#47602,#47603,#47604,#47605,#47606,#47607,#47608,#47609,#47610,
#47611,#47612,#47613,#47614,#47615,#47616,#47617,#47618,#47619,#47620,#47621,
#47622,#47623,#47624,#47625,#47626,#47627,#47628,#47629,#47630,#47631,#47632,
#47633,#47634,#47635,#47636,#47637,#47638,#47639,#47640,#47641,#47642,#47643,
#47644,#47645,#47646,#47647,#47648,#47649,#47650,#47651,#47652,#47653,#47654,
#47655,#47656,#47657,#47658,#47659,#47660,#47661,#47662,#47663,#47664,#47665,
#47666,#47667,#47668,#47669,#47670,#47671,#47672,#47673,#47674,#47675,#47676,
#47677,#47678,#47679,#47680,#47681,#47682,#47683,#47684,#47685,#47686,#47687,
#47688,#47689,#47690,#47691,#47692,#47693,#47694,#47695,#47696),
 .UNSPECIFIED.,.F.,.F.,(4,3,3,3,3,3,3,3,3,3,3,3,3,3,3,3,3,3,3,3,3,3,3,3,
3,3,3,3,3,3,3,3,3,3,3,3,3,3,3,3,3,4),(112.18179093325,112.280032836003,
112.378281939794,112.476633715995,112.575038453655,112.673614632877,112.749405680676,
112.84800380568,112.946461588456,113.046684156229,113.144963713957,113.24321029303,
113.341453376069,113.443150564711,113.54153497813,113.644888554384,113.748242130638,
113.846840255641,113.945298038418,114.045520606191,114.143800163919,114.242046742992,
114.340289826031,114.441987014673,114.540371428091,114.643725004345,114.747078580599,
114.845676705603,114.944134488379,115.044357056152,115.14263661388,115.240883192953,
115.339126275992,115.440823464634,115.539207878053,115.642561454307,115.745915030561,
115.84988875933,115.953561696348,116.057054365164,116.160309146371,116.238928182547),
 .UNSPECIFIED.);
#428=B_SPLINE_CURVE_WITH_KNOTS('',3,(#47697,#47698,#47699,#47700,#47701,
#47702,#47703,#47704,#47705,#47706,#47707,#47708,#47709,#47710,#47711,#47712,
#47713,#47714,#47715,#47716,#47717,#47718,#47719,#47720,#47721,#47722,#47723,
#47724,#47725,#47726,#47727,#47728,#47729,#47730,#47731,#47732,#47733,#47734,
#47735,#47736,#47737,#47738,#47739,#47740,#47741,#47742,#47743,#47744,#47745,
#47746,#47747,#47748,#47749,#47750,#47751,#47752,#47753,#47754,#47755,#47756,
#47757,#47758,#47759,#47760,#47761,#47762,#47763,#47764,#47765,#47766),
 .UNSPECIFIED.,.F.,.F.,(4,3,3,3,3,3,3,3,3,3,3,3,3,3,3,3,3,3,3,3,3,3,3,4),
(116.238928182823,116.341566510357,116.44447107289,116.547509821617,116.650828963887,
116.744751480523,116.843349605527,116.941807388303,117.042029956076,117.140309513804,
117.238556092878,117.336799175916,117.438496364558,117.536880777977,117.640234354231,
117.743587930485,117.842162082216,117.940606624238,118.038951269659,118.137225626952,
118.235476585644,118.333714612383,118.431998836546,118.464214608881),
 .UNSPECIFIED.);
#429=B_SPLINE_CURVE_WITH_KNOTS('',3,(#47768,#47769,#47770,#47771,#47772,
#47773,#47774,#47775,#47776,#47777,#47778,#47779,#47780,#47781,#47782,#47783,
#47784,#47785,#47786,#47787,#47788,#47789,#47790,#47791,#47792,#47793,#47794,
#47795,#47796,#47797,#47798,#47799,#47800,#47801,#47802,#47803,#47804,#47805,
#47806,#47807,#47808,#47809,#47810,#47811,#47812,#47813,#47814,#47815,#47816,
#47817,#47818,#47819,#47820,#47821,#47822,#47823,#47824,#47825,#47826,#47827,
#47828,#47829,#47830,#47831,#47832,#47833,#47834,#47835,#47836,#47837),
 .UNSPECIFIED.,.F.,.F.,(4,3,3,3,3,3,3,3,3,3,3,3,3,3,3,3,3,3,3,3,3,3,3,4),
(116.238928182823,116.279944748004,116.378542873008,116.477000655784,116.577223223557,
116.675502781285,116.773749360358,116.871992443397,116.973689632039,117.072074045458,
117.175427621712,117.278781197966,117.37737932297,117.475837105746,117.576059673519,
117.674339231247,117.77258581032,117.870828893359,117.972526082001,118.07091049542,
118.174264071673,118.277617647927,118.376189313834,118.465360150378),
 .UNSPECIFIED.);
#430=B_SPLINE_CURVE_WITH_KNOTS('',3,(#47838,#47839,#47840,#47841,#47842,
#47843,#47844,#47845),.UNSPECIFIED.,.F.,.F.,(4,1,1,1,1,4),(112.180986328742,
112.284598948156,113.283435398118,114.28227184808,115.281108298042,116.2389227975),
 .UNSPECIFIED.);
#431=B_SPLINE_CURVE_WITH_KNOTS('',3,(#47851,#47852,#47853,#47854,#47855,
#47856,#47857,#47858,#47859,#47860,#47861,#47862,#47863,#47864,#47865,#47866,
#47867,#47868,#47869,#47870,#47871,#47872,#47873,#47874,#47875,#47876,#47877,
#47878,#47879,#47880,#47881,#47882,#47883,#47884,#47885,#47886,#47887,#47888,
#47889,#47890,#47891,#47892,#47893,#47894,#47895,#47896,#47897,#47898,#47899,
#47900,#47901,#47902,#47903,#47904,#47905,#47906,#47907,#47908,#47909,#47910,
#47911,#47912,#47913,#47914,#47915,#47916,#47917,#47918,#47919,#47920,#47921,
#47922,#47923,#47924,#47925,#47926,#47927,#47928,#47929,#47930,#47931,#47932,
#47933,#47934,#47935,#47936,#47937,#47938,#47939,#47940,#47941,#47942,#47943,
#47944,#47945,#47946,#47947,#47948,#47949,#47950,#47951,#47952,#47953,#47954,
#47955,#47956,#47957,#47958,#47959,#47960,#47961,#47962,#47963,#47964,#47965,
#47966,#47967,#47968,#47969,#47970,#47971,#47972,#47973,#47974),
 .UNSPECIFIED.,.F.,.F.,(4,3,3,3,3,3,3,3,3,3,3,3,3,3,3,3,3,3,3,3,3,3,3,3,
3,3,3,3,3,3,3,3,3,3,3,3,3,3,3,3,3,4),(105.898938929587,105.99734597658,
106.095658484987,106.193920762289,106.292162310713,106.390412604461,106.488766496703,
106.587174737975,106.685752817441,106.756386980904,106.854985105908,106.953442888684,
107.053665456457,107.151945014185,107.250191593259,107.348434676297,107.450131864939,
107.548516278358,107.651869854612,107.755223430866,107.85382155587,107.952279338646,
108.052501906419,108.150781464147,108.249028043221,108.347271126259,108.448968314902,
108.54735272832,108.650706304574,108.754059880828,108.852658005832,108.951115788608,
109.051338356381,109.149617914109,109.247864493183,109.346107576221,109.447804764863,
109.546189178282,109.649542754536,109.75289633079,109.893212936358,109.955742875643),
 .UNSPECIFIED.);
#432=B_SPLINE_CURVE_WITH_KNOTS('',3,(#47975,#47976,#47977,#47978,#47979,
#47980,#47981,#47982,#47983,#47984,#47985,#47986,#47987,#47988,#47989,#47990,
#47991,#47992,#47993,#47994,#47995,#47996,#47997,#47998,#47999,#48000,#48001,
#48002,#48003,#48004,#48005,#48006,#48007,#48008,#48009,#48010,#48011,#48012,
#48013,#48014,#48015,#48016,#48017,#48018,#48019,#48020,#48021,#48022,#48023,
#48024,#48025,#48026,#48027,#48028,#48029,#48030,#48031,#48032,#48033,#48034,
#48035,#48036,#48037,#48038,#48039,#48040,#48041,#48042,#48043,#48044,#48045,
#48046,#48047),.UNSPECIFIED.,.F.,.F.,(4,3,3,3,3,3,3,3,3,3,3,3,3,3,3,3,3,
3,3,3,3,3,3,3,4),(109.955742875951,110.055241614051,110.152151423466,110.249014842069,
110.345862894414,110.447330365999,110.544300028994,110.641334438529,110.738518045248,
110.751732780752,110.850330905756,110.948788688532,111.049011256305,111.147290814033,
111.245537393107,111.343780476145,111.445477664787,111.543862078206,111.64721565446,
111.750569230714,111.849176820414,111.947618966285,112.045965736407,112.144240689691,
112.18179093325),.UNSPECIFIED.);
#433=B_SPLINE_CURVE_WITH_KNOTS('',3,(#48049,#48050,#48051,#48052,#48053,
#48054),.UNSPECIFIED.,.F.,.F.,(4,1,1,4),(109.955750010087,110.286926048232,
111.285762498194,112.180986328742),.UNSPECIFIED.);
#434=B_SPLINE_CURVE_WITH_KNOTS('',3,(#48055,#48056,#48057,#48058,#48059,
#48060,#48061,#48062,#48063,#48064,#48065,#48066,#48067,#48068,#48069,#48070,
#48071,#48072,#48073,#48074,#48075,#48076,#48077,#48078,#48079,#48080,#48081,
#48082,#48083,#48084,#48085,#48086,#48087,#48088,#48089,#48090,#48091,#48092,
#48093,#48094,#48095,#48096,#48097,#48098,#48099,#48100,#48101,#48102,#48103,
#48104,#48105,#48106,#48107,#48108,#48109,#48110,#48111,#48112,#48113,#48114,
#48115,#48116,#48117,#48118,#48119,#48120,#48121,#48122,#48123,#48124,#48125,
#48126,#48127,#48128,#48129,#48130,#48131,#48132,#48133,#48134,#48135,#48136,
#48137,#48138,#48139,#48140,#48141,#48142,#48143,#48144,#48145,#48146,#48147,
#48148,#48149,#48150,#48151,#48152,#48153,#48154,#48155,#48156,#48157,#48158,
#48159,#48160,#48161,#48162,#48163,#48164,#48165,#48166,#48167,#48168,#48169,
#48170,#48171,#48172,#48173,#48174,#48175,#48176,#48177,#48178),
 .UNSPECIFIED.,.F.,.F.,(4,3,3,3,3,3,3,3,3,3,3,3,3,3,3,3,3,3,3,3,3,3,3,3,
3,3,3,3,3,3,3,3,3,3,3,3,3,3,3,3,3,4),(105.898082546227,105.996456971766,
106.094847348914,106.193416319605,106.291580248385,106.390178373389,106.488636156165,
106.588858723938,106.687138281666,106.78538486074,106.883627943778,106.98532513242,
107.083709545839,107.187063122093,107.290416698347,107.389014823351,107.487472606128,
107.5876951739,107.685974731629,107.784221310702,107.882464393741,107.984161582383,
108.082545995802,108.185899572055,108.289253148309,108.387851273313,108.486309056089,
108.586531623862,108.68481118159,108.783057760664,108.881300843702,108.982998032345,
109.081382445763,109.184736022017,109.288089598271,109.386591328535,109.484956309733,
109.583214317042,109.681399820024,109.779540599734,109.877698313765,109.955742875643),
 .UNSPECIFIED.);
#435=B_SPLINE_CURVE_WITH_KNOTS('',3,(#48184,#48185,#48186,#48187,#48188,
#48189,#48190,#48191),.UNSPECIFIED.,.F.,.F.,(4,1,1,1,1,4),(99.6144332342635,
99.7645318311714,100.763368281133,101.762204731095,102.761041181057,103.672548858934),
 .UNSPECIFIED.);
#436=B_SPLINE_CURVE_WITH_KNOTS('',3,(#48192,#48193,#48194,#48195,#48196,
#48197,#48198,#48199,#48200,#48201,#48202,#48203,#48204,#48205,#48206,#48207,
#48208,#48209,#48210,#48211,#48212,#48213,#48214,#48215,#48216,#48217,#48218,
#48219,#48220,#48221,#48222,#48223,#48224,#48225,#48226,#48227,#48228,#48229,
#48230,#48231,#48232,#48233,#48234,#48235,#48236,#48237,#48238,#48239,#48240,
#48241,#48242,#48243,#48244,#48245,#48246,#48247,#48248,#48249,#48250,#48251,
#48252,#48253,#48254,#48255,#48256,#48257,#48258,#48259,#48260,#48261),
 .UNSPECIFIED.,.F.,.F.,(4,3,3,3,3,3,3,3,3,3,3,3,3,3,3,3,3,3,3,3,3,3,3,4),
(103.672557568463,103.759877631019,103.858475756023,103.9569335388,104.057156106572,
104.1554356643,104.253682243374,104.351925326412,104.453622515055,104.552006928473,
104.655360504727,104.758714080981,104.857312205985,104.955769988761,105.055992556534,
105.154272114262,105.252518693336,105.350761776374,105.452458965016,105.550843378435,
105.654196954689,105.757550530943,105.856140410584,105.898938929587),
 .UNSPECIFIED.);
#437=B_SPLINE_CURVE_WITH_KNOTS('',3,(#48263,#48264,#48265,#48266,#48267,
#48268,#48269,#48270,#48271,#48272,#48273,#48274,#48275,#48276,#48277,#48278,
#48279,#48280,#48281,#48282,#48283,#48284,#48285,#48286,#48287,#48288,#48289,
#48290,#48291,#48292,#48293,#48294,#48295,#48296,#48297,#48298,#48299,#48300,
#48301,#48302,#48303,#48304,#48305,#48306,#48307,#48308,#48309,#48310,#48311,
#48312,#48313,#48314,#48315,#48316,#48317,#48318,#48319,#48320,#48321,#48322,
#48323,#48324,#48325,#48326,#48327,#48328,#48329,#48330,#48331,#48332,#48333,
#48334,#48335),.UNSPECIFIED.,.F.,.F.,(4,3,3,3,3,3,3,3,3,3,3,3,3,3,3,3,3,
3,3,3,3,3,3,3,4),(103.672557568463,103.771601702603,103.870660322484,103.96976131202,
104.06899945985,104.168318657834,104.267812431338,104.293907348461,104.392505473465,
104.490963256242,104.591185824014,104.689465381742,104.787711960816,104.885955043854,
104.987652232497,105.086036645915,105.189390222169,105.292743798423,105.39132916073,
105.489781902009,105.591857063063,105.690131969833,105.788367325292,105.886604359629,
105.898082546227),.UNSPECIFIED.);
#438=B_SPLINE_CURVE_WITH_KNOTS('',3,(#48336,#48337,#48338,#48339,#48340,
#48341,#48342,#48343),.UNSPECIFIED.,.F.,.F.,(4,1,1,1,1,4),(99.6160278953699,
100.298561548614,101.297397998576,102.296234448537,103.295070898499,103.672550060693),
 .UNSPECIFIED.);
#439=B_SPLINE_CURVE_WITH_KNOTS('',3,(#48349,#48350,#48351,#48352,#48353,
#48354,#48355,#48356,#48357,#48358,#48359,#48360,#48361,#48362,#48363,#48364,
#48365,#48366,#48367,#48368,#48369,#48370,#48371,#48372,#48373,#48374,#48375,
#48376,#48377,#48378,#48379,#48380,#48381,#48382,#48383,#48384,#48385,#48386,
#48387,#48388,#48389,#48390,#48391,#48392,#48393,#48394,#48395,#48396,#48397,
#48398,#48399,#48400,#48401,#48402,#48403,#48404,#48405,#48406,#48407,#48408,
#48409,#48410,#48411,#48412,#48413,#48414,#48415,#48416,#48417,#48418,#48419,
#48420,#48421,#48422,#48423,#48424,#48425,#48426,#48427,#48428,#48429,#48430,
#48431,#48432,#48433,#48434,#48435,#48436,#48437,#48438,#48439,#48440,#48441,
#48442,#48443,#48444,#48445,#48446,#48447,#48448,#48449,#48450,#48451,#48452,
#48453,#48454,#48455,#48456,#48457,#48458,#48459,#48460,#48461,#48462,#48463,
#48464,#48465,#48466,#48467,#48468,#48469,#48470,#48471,#48472,#48473,#48474,
#48475),.UNSPECIFIED.,.F.,.F.,(4,3,3,3,3,3,3,3,3,3,3,3,3,3,3,3,3,3,3,3,
3,3,3,3,3,3,3,3,3,3,3,3,3,3,3,3,3,3,3,3,3,3,4),(93.3318434563844,93.4301005392899,
93.5284655236451,93.6268914765217,93.7254798512049,93.7715131314001,93.8701112564038,
93.9685690391806,94.0687916069533,94.1670711646814,94.2653177437548,94.3635608267931,
94.4652580154354,94.5636424288541,94.6669960051081,94.770349581362,94.8689477063657,
94.9674054891425,95.0676280569152,95.1659076146434,95.2641541937167,95.3623972767553,
95.4640944653975,95.5624788788163,95.6658324550701,95.7691860313239,95.8677841563277,
95.9662419391043,96.066464506877,96.1647440646051,96.2629906436786,96.3612337267171,
96.4629309153592,96.561315328778,96.6646689050319,96.7680224812857,96.867499372579,
96.9668292609829,97.0660403563902,97.1651524247998,97.264207533224,97.3632407686273,
97.3893722612837),.UNSPECIFIED.);
#440=B_SPLINE_CURVE_WITH_KNOTS('',3,(#48476,#48477,#48478,#48479,#48480,
#48481),.UNSPECIFIED.,.F.,.F.,(4,1,1,4),(97.389379769506,97.7668589312476,
98.7656953812095,99.6144332342635),.UNSPECIFIED.);
#441=B_SPLINE_CURVE_WITH_KNOTS('',3,(#48483,#48484,#48485,#48486,#48487,
#48488),.UNSPECIFIED.,.F.,.F.,(4,1,1,4),(97.3893809713061,98.3008886486899,
99.2997250986518,99.6160278953699),.UNSPECIFIED.);
#442=B_SPLINE_CURVE_WITH_KNOTS('',3,(#48489,#48490,#48491,#48492,#48493,
#48494,#48495,#48496,#48497,#48498,#48499,#48500,#48501,#48502,#48503,#48504,
#48505,#48506,#48507,#48508,#48509,#48510,#48511,#48512,#48513,#48514,#48515,
#48516,#48517,#48518,#48519,#48520,#48521,#48522,#48523,#48524,#48525,#48526,
#48527,#48528,#48529,#48530,#48531,#48532,#48533,#48534,#48535,#48536,#48537,
#48538,#48539,#48540,#48541,#48542,#48543,#48544,#48545,#48546,#48547,#48548,
#48549,#48550,#48551,#48552,#48553,#48554,#48555,#48556,#48557,#48558,#48559,
#48560,#48561,#48562,#48563,#48564,#48565,#48566,#48567,#48568,#48569,#48570,
#48571,#48572,#48573,#48574,#48575,#48576,#48577,#48578,#48579,#48580,#48581,
#48582,#48583,#48584,#48585,#48586,#48587,#48588,#48589,#48590,#48591,#48592,
#48593,#48594,#48595,#48596,#48597,#48598,#48599,#48600,#48601,#48602,#48603,
#48604,#48605,#48606,#48607,#48608,#48609,#48610,#48611,#48612),
 .UNSPECIFIED.,.F.,.F.,(4,3,3,3,3,3,3,3,3,3,3,3,3,3,3,3,3,3,3,3,3,3,3,3,
3,3,3,3,3,3,3,3,3,3,3,3,3,3,3,3,3,4),(93.3321733281741,93.4307320743328,
93.5291589655597,93.627483394628,93.7257523855544,93.8239954482649,93.9222420599768,
94.020589121044,94.1189858625401,94.2175579041604,94.3055428488424,94.4041409738461,
94.5025987566229,94.6028213243956,94.7011008821237,94.7993474611971,94.8975905442356,
94.9992877328778,95.0976721462966,95.2010257225505,95.3043792988043,95.402977423808,
95.5014352065847,95.6016577743574,95.6999373320855,95.7981839111589,95.8964269941973,
95.9981241828395,96.0965085962583,96.1998621725122,96.3032157487661,96.4018138737698,
96.5002716565465,96.6004942243192,96.6987737820473,96.7970203611207,96.8952634441592,
96.9969606328014,97.0953450462202,97.1986986224741,97.302052198728,97.3893722612837),
 .UNSPECIFIED.);
#443=B_SPLINE_CURVE_WITH_KNOTS('',3,(#48618,#48619,#48620,#48621,#48622,
#48623,#48624,#48625),.UNSPECIFIED.,.F.,.F.,(4,1,1,1,1,4),(87.0497429340083,
87.7784944316289,88.7773308815907,89.7761673315526,90.7750037815145,91.1061798190739),
 .UNSPECIFIED.);
#444=B_SPLINE_CURVE_WITH_KNOTS('',3,(#48626,#48627,#48628,#48629,#48630,
#48631,#48632,#48633,#48634,#48635,#48636,#48637,#48638,#48639,#48640,#48641,
#48642,#48643,#48644,#48645,#48646,#48647,#48648,#48649,#48650,#48651,#48652,
#48653,#48654,#48655,#48656,#48657,#48658,#48659,#48660,#48661,#48662,#48663,
#48664,#48665,#48666,#48667,#48668,#48669,#48670,#48671,#48672,#48673,#48674,
#48675,#48676,#48677,#48678,#48679,#48680,#48681,#48682,#48683,#48684,#48685,
#48686,#48687,#48688,#48689,#48690,#48691,#48692,#48693,#48694,#48695),
 .UNSPECIFIED.,.F.,.F.,(4,3,3,3,3,3,3,3,3,3,3,3,3,3,3,3,3,3,3,3,3,3,3,4),
(91.1061869541041,91.2043419644769,91.3024795334306,91.4006291648835,91.4988897541851,
91.5972075103073,91.6957053368608,91.7738402314764,91.8724383564801,91.9708961392569,
92.0711187070296,92.1693982647577,92.2676448438311,92.3658879268697,92.4675851155119,
92.5659695289307,92.6693231051844,92.7726766814382,92.8712673172517,92.9697241251225,
93.0680663331336,93.16634103844,93.2645927043654,93.3318434563844),
 .UNSPECIFIED.);
#445=B_SPLINE_CURVE_WITH_KNOTS('',3,(#48697,#48698,#48699,#48700,#48701,
#48702,#48703,#48704,#48705,#48706,#48707,#48708,#48709,#48710,#48711,#48712,
#48713,#48714,#48715,#48716,#48717,#48718,#48719,#48720,#48721,#48722,#48723,
#48724,#48725,#48726,#48727,#48728,#48729,#48730,#48731,#48732,#48733,#48734,
#48735,#48736,#48737,#48738,#48739,#48740,#48741,#48742,#48743,#48744,#48745,
#48746,#48747,#48748,#48749,#48750,#48751,#48752,#48753,#48754,#48755,#48756,
#48757,#48758,#48759,#48760,#48761,#48762,#48763,#48764,#48765,#48766),
 .UNSPECIFIED.,.F.,.F.,(4,3,3,3,3,3,3,3,3,3,3,3,3,3,3,3,3,3,3,3,3,3,3,4),
(91.1061869541041,91.2465035596788,91.3090334989568,91.4076316239605,91.5060894067373,
91.6063119745099,91.7045915322381,91.8028381113114,91.90108119435,92.0027783829921,
92.1011627964109,92.2045163726648,92.3078699489186,92.4064680739223,92.5049258566991,
92.6051484244718,92.7034279821999,92.8016745612734,92.8999176443119,93.001614832954,
93.0999992463728,93.2033528226267,93.3067063988805,93.3321733281741),
 .UNSPECIFIED.);
#446=B_SPLINE_CURVE_WITH_KNOTS('',3,(#48767,#48768,#48769,#48770,#48771,
#48772,#48773,#48774,#48775,#48776,#48777,#48778,#48779,#48780,#48781,#48782,
#48783,#48784,#48785,#48786,#48787,#48788,#48789,#48790,#48791,#48792,#48793,
#48794,#48795,#48796,#48797,#48798,#48799,#48800,#48801,#48802,#48803,#48804,
#48805,#48806,#48807,#48808,#48809,#48810,#48811,#48812,#48813,#48814,#48815,
#48816,#48817,#48818,#48819,#48820,#48821,#48822,#48823,#48824,#48825,#48826,
#48827,#48828,#48829,#48830,#48831,#48832,#48833,#48834,#48835,#48836,#48837,
#48838,#48839,#48840,#48841,#48842,#48843,#48844,#48845,#48846,#48847,#48848,
#48849,#48850,#48851,#48852,#48853,#48854,#48855,#48856,#48857,#48858,#48859,
#48860,#48861,#48862,#48863,#48864,#48865,#48866,#48867,#48868,#48869,#48870,
#48871,#48872,#48873,#48874,#48875,#48876,#48877,#48878,#48879,#48880,#48881,
#48882,#48883,#48884,#48885,#48886,#48887,#48888,#48889,#48890,#48891,#48892,
#48893),.UNSPECIFIED.,.F.,.F.,(4,3,3,3,3,3,3,3,3,3,3,3,3,3,3,3,3,3,3,3,
3,3,3,3,3,3,3,3,3,3,3,3,3,3,3,3,3,3,3,3,3,3,4),(87.0482730717182,87.1466828354347,
87.2452617559357,87.3136876991093,87.412285824113,87.5107436068897,87.6109661746624,
87.7092457323906,87.807492311464,87.9057353945024,88.0074325831446,88.1058169965634,
88.2091705728173,88.3125241490712,88.4111222740749,88.5095800568517,88.6098026246243,
88.7080821823525,88.8063287614258,88.9045718444643,89.0062690331065,89.1046534465253,
89.2080070227792,89.311360599033,89.4099587240367,89.5084165068134,89.6086390745861,
89.7069186323142,89.8051652113876,89.9034082944261,90.0051054830683,90.1034898964871,
90.206843472741,90.3101970489949,90.409695787095,90.5067185530535,90.6036495481492,
90.70051989818,90.801936662084,90.8988156754798,90.9957205549588,91.0927209416413,
91.1061869537961),.UNSPECIFIED.);
#447=B_SPLINE_CURVE_WITH_KNOTS('',3,(#48899,#48900,#48901,#48902,#48903,
#48904,#48905,#48906,#48907,#48908,#48909,#48910,#48911,#48912,#48913,#48914,
#48915,#48916,#48917,#48918,#48919,#48920,#48921,#48922,#48923,#48924,#48925,
#48926,#48927,#48928,#48929,#48930,#48931,#48932,#48933,#48934,#48935,#48936,
#48937,#48938,#48939,#48940,#48941,#48942,#48943,#48944,#48945,#48946,#48947,
#48948,#48949,#48950,#48951,#48952,#48953,#48954,#48955,#48956,#48957,#48958,
#48959,#48960,#48961,#48962,#48963,#48964,#48965,#48966,#48967,#48968,#48969,
#48970,#48971,#48972,#48973,#48974,#48975,#48976,#48977,#48978,#48979,#48980,
#48981,#48982,#48983,#48984,#48985,#48986,#48987,#48988,#48989,#48990,#48991,
#48992,#48993,#48994,#48995,#48996,#48997,#48998,#48999,#49000,#49001,#49002,
#49003,#49004,#49005,#49006,#49007,#49008,#49009,#49010,#49011,#49012,#49013,
#49014,#49015,#49016,#49017,#49018,#49019,#49020,#49021,#49022,#49023,#49024,
#49025),.UNSPECIFIED.,.F.,.F.,(4,3,3,3,3,3,3,3,3,3,3,3,3,3,3,3,3,3,3,3,
3,3,3,3,3,3,3,3,3,3,3,3,3,3,3,3,3,3,3,3,3,3,4),(80.7655329641705,80.7866392818957,
80.8852374068994,80.9836951896762,81.0839177574489,81.182197315177,81.2804438942504,
81.3786869772889,81.4803841659311,81.5787685793499,81.6821221556037,81.7854757318576,
81.8840738568613,81.982531639638,82.0827542074107,82.1810337651389,82.2792803442123,
82.3775234272508,82.4792206158929,82.5776050293117,82.6809586055656,82.7843121818195,
82.8829103068232,82.9813680896,83.0815906573726,83.1798702151008,83.2781167941742,
83.3763598772127,83.4780570658549,83.5764414792737,83.6797950555275,83.7831486317814,
83.8817467567851,83.9802045395617,84.0804271073344,84.1787066650626,84.276953244136,
84.3751963271744,84.4768935158166,84.5752779292354,84.6786315054893,84.7819850817432,
84.8230016469246),.UNSPECIFIED.);
#448=B_SPLINE_CURVE_WITH_KNOTS('',3,(#49026,#49027,#49028,#49029,#49030,
#49031),.UNSPECIFIED.,.F.,.F.,(4,1,1,4),(84.8230070319889,85.7808215317051,
86.779657981667,87.0497429340083),.UNSPECIFIED.);
#449=B_SPLINE_CURVE_WITH_KNOTS('',3,(#49033,#49034,#49035,#49036,#49037,
#49038,#49039,#49040,#49041,#49042,#49043,#49044,#49045,#49046,#49047,#49048,
#49049,#49050,#49051,#49052,#49053,#49054,#49055,#49056,#49057,#49058,#49059,
#49060,#49061,#49062,#49063,#49064,#49065,#49066,#49067,#49068,#49069,#49070,
#49071,#49072,#49073,#49074,#49075,#49076,#49077,#49078,#49079,#49080,#49081,
#49082,#49083,#49084,#49085,#49086,#49087,#49088,#49089,#49090,#49091,#49092,
#49093,#49094,#49095,#49096,#49097,#49098,#49099,#49100,#49101,#49102),
 .UNSPECIFIED.,.F.,.F.,(4,3,3,3,3,3,3,3,3,3,3,3,3,3,3,3,3,3,3,3,3,3,3,4),
(84.8230016472006,84.9261861619503,85.029664796698,85.133294590709,85.2372126194223,
85.3160147991855,85.4146129241892,85.513070706966,85.6132932747387,85.7115728324668,
85.8098194115402,85.9080624945788,86.0097596832209,86.1081440966398,86.2114976728936,
86.3148512491474,86.4134243290379,86.5118681332251,86.6102123732651,86.7084866565464,
86.8067399239172,86.9049803913521,87.003272709464,87.0482730717182),
 .UNSPECIFIED.);
#450=B_SPLINE_CURVE_WITH_KNOTS('',3,(#49103,#49104,#49105,#49106,#49107,
#49108,#49109,#49110,#49111,#49112,#49113,#49114,#49115,#49116,#49117,#49118,
#49119,#49120,#49121,#49122,#49123,#49124,#49125,#49126,#49127,#49128,#49129,
#49130,#49131,#49132,#49133,#49134,#49135,#49136,#49137,#49138,#49139,#49140,
#49141,#49142,#49143,#49144,#49145,#49146,#49147,#49148,#49149,#49150,#49151,
#49152,#49153,#49154,#49155,#49156,#49157,#49158,#49159,#49160,#49161,#49162,
#49163,#49164,#49165,#49166,#49167,#49168,#49169,#49170,#49171,#49172,#49173,
#49174,#49175,#49176,#49177,#49178,#49179,#49180,#49181,#49182,#49183,#49184,
#49185,#49186,#49187,#49188,#49189,#49190,#49191,#49192,#49193,#49194,#49195,
#49196,#49197,#49198,#49199,#49200,#49201,#49202,#49203,#49204,#49205,#49206,
#49207,#49208,#49209,#49210,#49211,#49212,#49213,#49214,#49215,#49216,#49217,
#49218,#49219,#49220,#49221,#49222,#49223,#49224,#49225,#49226),
 .UNSPECIFIED.,.F.,.F.,(4,3,3,3,3,3,3,3,3,3,3,3,3,3,3,3,3,3,3,3,3,3,3,3,
3,3,3,3,3,3,3,3,3,3,3,3,3,3,3,3,3,4),(80.7658264823238,80.8640676547198,
80.9623198591735,81.0606770182082,81.1590905811291,81.2576716388607,81.320668999338,
81.4192671243417,81.5177249071185,81.6179474748912,81.7162270326193,81.8144736116927,
81.9127166947311,82.0144138833733,82.1127982967922,82.216151873046,82.3195054492999,
82.4181035743036,82.5165613570806,82.6167839248532,82.7150634825814,82.8133100616548,
82.9115531446933,83.0132503333354,83.1116347467542,83.214988323008,83.3183418992618,
83.4169400242655,83.5153978070425,83.6156203748152,83.7138999325434,83.8121465116168,
83.9103895946552,84.0120867832973,84.1104711967161,84.2138247729699,84.3171783492237,
84.420557830251,84.523654386749,84.6265834813182,84.7292989065994,84.8230016469246),
 .UNSPECIFIED.);
#451=B_SPLINE_CURVE_WITH_KNOTS('',3,(#49232,#49233,#49234,#49235,#49236,
#49237,#49238,#49239),.UNSPECIFIED.,.F.,.F.,(4,1,1,1,1,4),(74.4816441296696,
74.7936205821245,75.7924570320864,76.7912934820482,77.7901299320101,78.539816339745),
 .UNSPECIFIED.);
#452=B_SPLINE_CURVE_WITH_KNOTS('',3,(#49240,#49241,#49242,#49243,#49244,
#49245,#49246,#49247,#49248,#49249,#49250,#49251,#49252,#49253,#49254,#49255,
#49256,#49257,#49258,#49259,#49260,#49261,#49262,#49263,#49264,#49265,#49266,
#49267,#49268,#49269,#49270,#49271,#49272,#49273,#49274,#49275,#49276,#49277,
#49278,#49279,#49280,#49281,#49282,#49283,#49284,#49285,#49286,#49287,#49288,
#49289,#49290,#49291,#49292,#49293,#49294,#49295,#49296,#49297,#49298,#49299,
#49300,#49301,#49302,#49303,#49304,#49305,#49306),.UNSPECIFIED.,.F.,.F.,
(4,3,3,3,3,3,3,3,3,3,3,3,3,3,3,3,3,3,3,3,3,3,4),(78.5398164398184,78.6677108218573,
78.788966381972,78.8875645069757,78.9860222897524,79.0862448575251,79.1845244152533,
79.2827709943266,79.3810140773651,79.4827112660073,79.5810956794261,79.68444925568,
79.7878028319339,79.8864023576699,79.9848611556885,80.0832042043516,80.1814836418339,
80.2797289912675,80.3779697355309,80.4762993937765,80.5746716764702,80.6732109328371,
80.7655329641705),.UNSPECIFIED.);
#453=B_SPLINE_CURVE_WITH_KNOTS('',3,(#49308,#49309,#49310,#49311,#49312,
#49313,#49314,#49315,#49316,#49317,#49318,#49319,#49320,#49321,#49322,#49323,
#49324,#49325,#49326,#49327,#49328,#49329,#49330,#49331,#49332,#49333,#49334,
#49335,#49336,#49337,#49338,#49339,#49340,#49341,#49342,#49343,#49344,#49345,
#49346,#49347,#49348,#49349,#49350,#49351,#49352,#49353,#49354,#49355,#49356,
#49357,#49358,#49359,#49360,#49361,#49362,#49363,#49364,#49365,#49366,#49367,
#49368,#49369,#49370,#49371,#49372,#49373,#49374,#49375,#49376,#49377),
 .UNSPECIFIED.,.F.,.F.,(4,3,3,3,3,3,3,3,3,3,3,3,3,3,3,3,3,3,3,3,3,3,3,4),
(78.539816339745,78.6377138097037,78.7346673304385,78.831578691398,78.9284788661294,
79.0271081744506,79.1241353185128,79.2235657089636,79.3229960994143,79.4215942244181,
79.5200520071948,79.6202745749675,79.7185541326956,79.816800711769,79.9150437948075,
80.0167409834497,80.1151253968684,80.2184789731223,80.3218325493762,80.4204382921282,
80.5188792313131,80.6172249291316,80.7155010605353,80.7658264823238),
 .UNSPECIFIED.);
#454=B_SPLINE_CURVE_WITH_KNOTS('',3,(#49378,#49379,#49380,#49381,#49382,
#49383,#49384,#49385),.UNSPECIFIED.,.F.,.F.,(4,1,1,1,1,4),(74.48326306339,
75.3276502995668,76.3264867495287,77.3253231994905,78.3241596494524,78.539816339745),
 .UNSPECIFIED.);
#455=B_SPLINE_CURVE_WITH_KNOTS('',3,(#49391,#49392,#49393,#49394,#49395,
#49396,#49397,#49398,#49399,#49400,#49401,#49402,#49403,#49404,#49405,#49406,
#49407,#49408,#49409,#49410,#49411,#49412,#49413,#49414,#49415,#49416,#49417,
#49418,#49419,#49420,#49421,#49422,#49423,#49424,#49425,#49426,#49427,#49428,
#49429,#49430,#49431,#49432,#49433,#49434,#49435,#49436,#49437,#49438,#49439,
#49440,#49441,#49442,#49443,#49444,#49445,#49446,#49447,#49448,#49449,#49450,
#49451,#49452,#49453,#49454,#49455,#49456,#49457,#49458,#49459,#49460,#49461,
#49462,#49463,#49464,#49465,#49466,#49467,#49468,#49469,#49470,#49471,#49472,
#49473,#49474,#49475,#49476,#49477,#49478,#49479,#49480,#49481,#49482,#49483,
#49484,#49485,#49486,#49487,#49488,#49489,#49490,#49491,#49492,#49493,#49494,
#49495,#49496,#49497,#49498,#49499,#49500,#49501,#49502,#49503,#49504,#49505,
#49506,#49507,#49508,#49509,#49510,#49511,#49512,#49513,#49514),
 .UNSPECIFIED.,.F.,.F.,(4,3,3,3,3,3,3,3,3,3,3,3,3,3,3,3,3,3,3,3,3,3,3,3,
3,3,3,3,3,3,3,3,3,3,3,3,3,3,3,3,3,4),(68.1995885950359,68.2978347616174,
68.3960781115758,68.4972090542702,68.595594464771,68.6980981735621,68.8006018823532,
68.8992000073568,68.9976577901334,69.0978803579061,69.1961599156343,69.2944064947077,
69.3926495777462,69.4943467663884,69.5927311798071,69.6960847560611,69.7994383323151,
69.8980364573188,69.9964942400959,70.0967168078685,70.1949963655966,70.29324294467,
70.3914860277084,70.4931832163506,70.5915676297695,70.6949212060232,70.798274782277,
70.8968729072807,70.9953306900577,71.0955532578304,71.1938328155586,71.292079394632,
71.3903224776701,71.4920196663123,71.5904040797311,71.693757655985,71.7971112322389,
71.9028340905511,72.0081993817375,72.1133399321499,72.2181701837239,72.2566308185779),
 .UNSPECIFIED.);
#456=B_SPLINE_CURVE_WITH_KNOTS('',3,(#49515,#49516,#49517,#49518,#49519,
#49520),.UNSPECIFIED.,.F.,.F.,(4,1,1,4),(72.2566310325654,72.7959476822007,
73.7947841321626,74.4816441296696),.UNSPECIFIED.);
#457=B_SPLINE_CURVE_WITH_KNOTS('',3,(#49522,#49523,#49524,#49525,#49526,
#49527,#49528),.UNSPECIFIED.,.F.,.F.,(4,1,1,1,4),(72.2566310325654,72.3311409496812,
73.329977399643,74.3288138496049,74.48326306339),.UNSPECIFIED.);
#458=B_SPLINE_CURVE_WITH_KNOTS('',3,(#49529,#49530,#49531,#49532,#49533,
#49534,#49535,#49536,#49537,#49538,#49539,#49540,#49541,#49542,#49543,#49544,
#49545,#49546,#49547,#49548,#49549,#49550,#49551,#49552,#49553,#49554,#49555,
#49556,#49557,#49558,#49559,#49560,#49561,#49562,#49563,#49564,#49565,#49566,
#49567,#49568,#49569,#49570,#49571,#49572,#49573,#49574,#49575,#49576,#49577,
#49578,#49579,#49580,#49581,#49582,#49583,#49584,#49585,#49586,#49587,#49588,
#49589,#49590,#49591,#49592,#49593,#49594,#49595,#49596,#49597,#49598,#49599,
#49600,#49601,#49602,#49603,#49604,#49605,#49606,#49607,#49608,#49609,#49610,
#49611,#49612,#49613,#49614,#49615,#49616,#49617,#49618,#49619,#49620,#49621,
#49622,#49623,#49624,#49625,#49626,#49627,#49628,#49629,#49630,#49631,#49632,
#49633,#49634,#49635,#49636,#49637,#49638,#49639,#49640,#49641,#49642,#49643,
#49644,#49645,#49646,#49647,#49648,#49649,#49650,#49651,#49652,#49653,#49654,
#49655),.UNSPECIFIED.,.F.,.F.,(4,3,3,3,3,3,3,3,3,3,3,3,3,3,3,3,3,3,3,3,
3,3,3,3,3,3,3,3,3,3,3,3,3,3,3,3,3,3,3,3,3,3,4),(68.1987515094134,68.2973434667343,
68.3357951498337,68.4343932748374,68.5328510576141,68.6330736253868,68.7313531831149,
68.8295997621883,68.9278428452268,69.029540033869,69.1279244472877,69.2312780235416,
69.3346315997955,69.4332297247992,69.5316875075759,69.6319100753486,69.7301896330768,
69.8284362121502,69.9266792951887,70.0283764838308,70.1267608972497,70.2301144735035,
70.3334680497574,70.4320661747611,70.5305239575378,70.6307465253105,70.7290260830386,
70.827272662112,70.9255157451505,71.0272129337927,71.1255973472115,71.2289509234654,
71.3323044997193,71.4298807240688,71.5273176349421,71.6246428433669,71.721908115062,
71.8191441424516,71.9163815796695,72.013708783522,72.1110862397604,72.2086145464311,
72.2566310325654),.UNSPECIFIED.);
#459=B_SPLINE_CURVE_WITH_KNOTS('',3,(#49661,#49662,#49663,#49664,#49665,
#49666,#49667,#49668),.UNSPECIFIED.,.F.,.F.,(4,1,1,1,1,4),(61.9167164919525,
62.807583182582,63.8064196325439,64.8052560825058,65.8040925324676,65.9734457253857),
 .UNSPECIFIED.);
#460=B_SPLINE_CURVE_WITH_KNOTS('',3,(#49669,#49670,#49671,#49672,#49673,
#49674,#49675,#49676,#49677,#49678,#49679,#49680,#49681,#49682,#49683,#49684,
#49685,#49686,#49687,#49688,#49689,#49690,#49691,#49692,#49693,#49694,#49695,
#49696,#49697,#49698,#49699,#49700,#49701,#49702,#49703,#49704,#49705,#49706,
#49707,#49708,#49709,#49710,#49711,#49712,#49713,#49714,#49715,#49716,#49717,
#49718,#49719,#49720,#49721,#49722,#49723,#49724,#49725,#49726,#49727,#49728,
#49729,#49730,#49731,#49732,#49733,#49734,#49735,#49736,#49737,#49738),
 .UNSPECIFIED.,.F.,.F.,(4,3,3,3,3,3,3,3,3,3,3,3,3,3,3,3,3,3,3,3,3,3,3,4),
(65.9734457253857,66.0704340596177,66.1673127975357,66.2641328887558,66.3609254267909,
66.4577214670338,66.5546134226801,66.6515579893416,66.7486626585398,66.8029289824295,
66.9015271074333,66.9999848902101,67.1002074579827,67.1984870157109,67.2967335947843,
67.3949766778227,67.4966738664648,67.5950582798836,67.6984118561375,67.8017654323914,
67.9012212230525,67.9996662408954,68.0996274179656,68.1995885950359),
 .UNSPECIFIED.);
#461=B_SPLINE_CURVE_WITH_KNOTS('',3,(#49740,#49741,#49742,#49743,#49744,
#49745,#49746,#49747,#49748,#49749,#49750,#49751,#49752,#49753,#49754,#49755,
#49756,#49757,#49758,#49759,#49760,#49761,#49762,#49763,#49764,#49765,#49766,
#49767,#49768,#49769,#49770,#49771,#49772,#49773,#49774,#49775,#49776,#49777,
#49778,#49779,#49780,#49781,#49782,#49783,#49784,#49785,#49786,#49787,#49788,
#49789,#49790,#49791,#49792,#49793,#49794,#49795,#49796,#49797,#49798,#49799,
#49800,#49801,#49802,#49803,#49804,#49805,#49806,#49807,#49808,#49809),
 .UNSPECIFIED.,.F.,.F.,(4,3,3,3,3,3,3,3,3,3,3,3,3,3,3,3,3,3,3,3,3,3,3,4),
(65.9734457256204,66.0848798050741,66.1968635637043,66.309495782683,66.3381222499099,
66.4367203749136,66.5351781576904,66.6354007254631,66.7336802831912,66.8319268622647,
66.9301699453032,67.0318671339453,67.1302515473642,67.233605123618,67.3369586998718,
67.4355663370597,67.5340045943449,67.6323466348068,67.7306220560096,67.828860384381,
67.9271329658739,68.0254205103649,68.1238183935028,68.1987515094134),
 .UNSPECIFIED.);
#462=B_SPLINE_CURVE_WITH_KNOTS('',3,(#49810,#49811,#49812,#49813,#49814,
#49815,#49816,#49817,#49818,#49819,#49820,#49821,#49822,#49823,#49824,#49825,
#49826,#49827,#49828,#49829,#49830,#49831,#49832,#49833,#49834,#49835,#49836,
#49837,#49838,#49839,#49840,#49841,#49842,#49843,#49844,#49845,#49846,#49847,
#49848,#49849,#49850,#49851,#49852,#49853,#49854,#49855,#49856,#49857,#49858,
#49859,#49860,#49861,#49862,#49863,#49864,#49865,#49866,#49867,#49868,#49869,
#49870,#49871,#49872,#49873,#49874,#49875,#49876,#49877,#49878,#49879,#49880,
#49881,#49882,#49883,#49884,#49885,#49886,#49887,#49888,#49889,#49890,#49891,
#49892,#49893,#49894,#49895,#49896,#49897,#49898,#49899,#49900,#49901,#49902,
#49903,#49904,#49905,#49906,#49907,#49908,#49909,#49910,#49911,#49912,#49913,
#49914,#49915,#49916,#49917,#49918,#49919,#49920,#49921,#49922,#49923,#49924,
#49925,#49926,#49927,#49928,#49929,#49930,#49931,#49932,#49933,#49934,#49935,
#49936),.UNSPECIFIED.,.F.,.F.,(4,3,3,3,3,3,3,3,3,3,3,3,3,3,3,3,3,3,3,3,
3,3,3,3,3,3,3,3,3,3,3,3,3,3,3,3,3,3,3,3,3,3,4),(61.9158792692003,62.0141406113804,
62.1125120186739,62.2109478385454,62.3095423735334,62.3427764500624,62.4413745750661,
62.5398323578429,62.6400549256156,62.7383344833437,62.8365810624171,62.9348241454556,
63.0365213340978,63.1349057475167,63.2382593237705,63.3416129000243,63.440211025028,
63.5386688078047,63.6388913755774,63.7371709333055,63.835417512379,63.9336605954173,
64.0353577840595,64.1337421974783,64.2370957737322,64.3404493499862,64.43904747499,
64.5375052577664,64.6377278255391,64.7360073832672,64.8342539623404,64.9324970453787,
65.0341942340211,65.1325786474399,65.235932223694,65.339285799948,65.4384637976082,
65.53749807745,65.6364173808604,65.7352455972605,65.8340208922139,65.932784900221,
65.9734457253857),.UNSPECIFIED.);
#463=B_SPLINE_CURVE_WITH_KNOTS('',3,(#49942,#49943,#49944,#49945,#49946,
#49947,#49948,#49949,#49950,#49951,#49952,#49953,#49954,#49955,#49956,#49957,
#49958,#49959,#49960,#49961,#49962,#49963,#49964,#49965,#49966,#49967,#49968,
#49969,#49970,#49971,#49972,#49973,#49974,#49975,#49976,#49977,#49978,#49979,
#49980,#49981,#49982,#49983,#49984,#49985,#49986,#49987,#49988,#49989,#49990,
#49991,#49992,#49993,#49994,#49995,#49996,#49997,#49998,#49999,#50000,#50001,
#50002,#50003,#50004,#50005,#50006,#50007,#50008,#50009,#50010,#50011,#50012,
#50013,#50014,#50015,#50016,#50017,#50018,#50019,#50020,#50021,#50022,#50023,
#50024,#50025,#50026,#50027,#50028,#50029,#50030,#50031,#50032,#50033,#50034,
#50035,#50036,#50037,#50038,#50039,#50040,#50041,#50042,#50043,#50044,#50045,
#50046,#50047,#50048,#50049,#50050,#50051,#50052,#50053,#50054,#50055,#50056,
#50057,#50058,#50059,#50060,#50061,#50062,#50063,#50064,#50065),
 .UNSPECIFIED.,.F.,.F.,(4,3,3,3,3,3,3,3,3,3,3,3,3,3,3,3,3,3,3,3,3,3,3,3,
3,3,3,3,3,3,3,3,3,3,3,3,3,3,3,3,3,4),(55.6323252039848,55.7308982682604,
55.8157280328489,55.9143261578526,56.0127839406293,56.113006508402,56.2112860661301,
56.3095326452035,56.407775728242,56.5094729168842,56.607857330303,56.7112109065569,
56.8145644828108,56.9131626078145,57.0116203905912,57.1118429583639,57.2101225160921,
57.3083690951655,57.4066121782039,57.5083093668461,57.6066937802649,57.7100473565188,
57.8134009327726,57.9119990577763,58.010456840553,58.1106794083257,58.2089589660538,
58.3072055451272,58.4054486281657,58.5071458168079,58.6055302302267,58.7088838064806,
58.8122373827345,58.9094791608007,59.0070768179764,59.1040671063404,59.2009981633325,
59.2979009849178,59.3959908432399,59.4929780422907,59.5916192302484,59.6902604182062),
 .UNSPECIFIED.);
#464=B_SPLINE_CURVE_WITH_KNOTS('',3,(#50066,#50067,#50068,#50069,#50070,
#50071,#50072),.UNSPECIFIED.,.F.,.F.,(4,1,1,1,4),(59.6902604182062,59.8110738326964,
60.8099102826583,61.8087467326201,61.9167164919525),.UNSPECIFIED.);
#465=B_SPLINE_CURVE_WITH_KNOTS('',3,(#50074,#50075,#50076,#50077,#50078,
#50079,#50080,#50081,#50082,#50083,#50084,#50085,#50086,#50087,#50088,#50089,
#50090,#50091,#50092,#50093,#50094,#50095,#50096,#50097,#50098,#50099,#50100,
#50101,#50102,#50103,#50104,#50105,#50106,#50107,#50108,#50109,#50110,#50111,
#50112,#50113,#50114,#50115,#50116,#50117,#50118,#50119,#50120,#50121,#50122,
#50123,#50124,#50125,#50126,#50127,#50128,#50129,#50130,#50131,#50132,#50133,
#50134,#50135,#50136,#50137,#50138,#50139,#50140,#50141,#50142,#50143),
 .UNSPECIFIED.,.F.,.F.,(4,3,3,3,3,3,3,3,3,3,3,3,3,3,3,3,3,3,3,3,3,3,3,4),
(59.6902604182062,59.7886341730559,59.8869985815967,59.985382791999,60.0838846667639,
60.182449929213,60.2811933482967,60.3451035501387,60.4437016751424,60.5421594579193,
60.6423820256919,60.74066158342,60.8389081624934,60.9371512455319,61.038848434174,
61.1372328475928,61.2405864238467,61.3439400001005,61.4425291322752,61.5409847704257,
61.6393272818741,61.7376024228517,61.8358589218591,61.9158792692003),
 .UNSPECIFIED.);
#466=B_SPLINE_CURVE_WITH_KNOTS('',3,(#50144,#50145,#50146,#50147,#50148,
#50149,#50150,#50151,#50152,#50153,#50154,#50155,#50156,#50157,#50158,#50159,
#50160,#50161,#50162,#50163,#50164,#50165,#50166,#50167,#50168,#50169,#50170,
#50171,#50172,#50173,#50174,#50175,#50176,#50177,#50178,#50179,#50180,#50181,
#50182,#50183,#50184,#50185,#50186,#50187,#50188,#50189,#50190,#50191,#50192,
#50193,#50194,#50195,#50196,#50197,#50198,#50199,#50200,#50201,#50202,#50203,
#50204,#50205,#50206,#50207,#50208,#50209,#50210,#50211,#50212,#50213,#50214,
#50215,#50216,#50217,#50218,#50219,#50220,#50221,#50222,#50223,#50224,#50225,
#50226,#50227,#50228,#50229,#50230,#50231,#50232,#50233,#50234,#50235,#50236,
#50237,#50238,#50239,#50240,#50241,#50242,#50243,#50244,#50245,#50246,#50247,
#50248,#50249,#50250,#50251,#50252,#50253,#50254,#50255,#50256,#50257,#50258,
#50259,#50260,#50261,#50262,#50263,#50264,#50265,#50266,#50267),
 .UNSPECIFIED.,.F.,.F.,(4,3,3,3,3,3,3,3,3,3,3,3,3,3,3,3,3,3,3,3,3,3,3,3,
3,3,3,3,3,3,3,3,3,3,3,3,3,3,3,3,3,4),(55.6334625497945,55.7317495942871,
55.8299992378273,55.9282409671961,56.0265042526908,56.1248784994769,56.2233186098339,
56.3219159047901,56.3497577502912,56.4483558752948,56.5468136580714,56.6470362258441,
56.7453157835723,56.8435623626456,56.9418054456839,57.0435026343262,57.141887047745,
57.245240623999,57.348594200253,57.4471923252566,57.5456501080335,57.6458726758062,
57.7441522335342,57.8423988126075,57.9406418956461,58.0423390842883,58.1407234977071,
58.244077073961,58.3474306502149,58.4460287752185,58.5444865579957,58.6447091257683,
58.7429886834964,58.8412352625698,58.9394783456081,59.0411755342503,59.1395599476692,
59.242913523923,59.3462671001768,59.4608829140302,59.5755716660047,59.6902604179793),
 .UNSPECIFIED.);
#467=B_SPLINE_CURVE_WITH_KNOTS('',3,(#50273,#50274,#50275,#50276,#50277,
#50278,#50279,#50280),.UNSPECIFIED.,.F.,.F.,(4,1,1,1,1,4),(49.3495871973939,
49.8227093330776,50.8215457830395,51.8203822330014,52.8192186829633,53.4070751110266),
 .UNSPECIFIED.);
#468=B_SPLINE_CURVE_WITH_KNOTS('',3,(#50281,#50282,#50283,#50284,#50285,
#50286,#50287,#50288,#50289,#50290,#50291,#50292,#50293,#50294,#50295,#50296,
#50297,#50298,#50299,#50300,#50301,#50302,#50303,#50304,#50305,#50306,#50307,
#50308,#50309,#50310,#50311,#50312,#50313,#50314,#50315,#50316,#50317,#50318,
#50319,#50320,#50321,#50322,#50323,#50324,#50325,#50326,#50327,#50328,#50329,
#50330,#50331,#50332,#50333,#50334,#50335,#50336,#50337,#50338,#50339,#50340,
#50341,#50342,#50343,#50344,#50345,#50346,#50347,#50348,#50349,#50350),
 .UNSPECIFIED.,.F.,.F.,(4,3,3,3,3,3,3,3,3,3,3,3,3,3,3,3,3,3,3,3,3,3,3,4),
(53.4070755243672,53.5149520672774,53.6231638610727,53.7318758460234,53.8180551329251,
53.9166532579288,54.0151110407056,54.1153336084783,54.2136131662065,54.3118597452798,
54.4101028283184,54.5118000169606,54.6101844303794,54.7135380066332,54.816891582887,
54.9188207855242,55.0172568627063,55.1155965180651,55.2138693495665,55.3121048834225,
55.4103643248623,55.5086391375978,55.6069975898681,55.6323252039848),
 .UNSPECIFIED.);
#469=B_SPLINE_CURVE_WITH_KNOTS('',3,(#50352,#50353,#50354,#50355,#50356,
#50357,#50358,#50359,#50360,#50361,#50362,#50363,#50364,#50365,#50366,#50367,
#50368,#50369,#50370,#50371,#50372,#50373,#50374,#50375,#50376,#50377,#50378,
#50379,#50380,#50381,#50382,#50383,#50384,#50385,#50386,#50387,#50388,#50389,
#50390,#50391,#50392,#50393,#50394,#50395,#50396,#50397,#50398,#50399,#50400,
#50401,#50402,#50403,#50404,#50405,#50406,#50407,#50408,#50409,#50410,#50411,
#50412,#50413,#50414,#50415,#50416,#50417,#50418,#50419,#50420,#50421),
 .UNSPECIFIED.,.F.,.F.,(4,3,3,3,3,3,3,3,3,3,3,3,3,3,3,3,3,3,3,3,3,3,3,4),
(53.4070751110266,53.5048543854907,53.602498370777,53.7000367768844,53.7975186210123,
53.894974367796,53.9924344477701,54.0899931990352,54.1876041339862,54.2853815723757,
54.3520848503674,54.4506829753711,54.5491407581478,54.6493633259204,54.7476428836486,
54.8458894627221,54.9441325457606,55.0458297344028,55.1442141478216,55.2475677240754,
55.3509213003293,55.4495112354527,55.5479503969119,55.6334625497945),
 .UNSPECIFIED.);
#470=B_SPLINE_CURVE_WITH_KNOTS('',3,(#50422,#50423,#50424,#50425,#50426,
#50427,#50428,#50429,#50430),.UNSPECIFIED.,.F.,.F.,(4,1,1,1,1,1,4),(49.3496771194667,
49.3579026005581,50.3567390505199,51.3555755004818,52.3544119504437,53.3532484004055,
53.4070751110266),.UNSPECIFIED.);
#471=B_SPLINE_CURVE_WITH_KNOTS('',3,(#50436,#50437,#50438,#50439,#50440,
#50441,#50442,#50443,#50444,#50445,#50446,#50447,#50448,#50449,#50450,#50451,
#50452,#50453,#50454,#50455,#50456,#50457,#50458,#50459,#50460,#50461,#50462,
#50463,#50464,#50465,#50466,#50467,#50468,#50469,#50470,#50471,#50472,#50473,
#50474,#50475,#50476,#50477,#50478,#50479,#50480,#50481,#50482,#50483,#50484,
#50485,#50486,#50487,#50488,#50489,#50490,#50491,#50492,#50493,#50494,#50495,
#50496,#50497,#50498,#50499,#50500,#50501,#50502,#50503,#50504,#50505,#50506,
#50507,#50508,#50509,#50510,#50511,#50512,#50513,#50514,#50515,#50516,#50517,
#50518,#50519,#50520,#50521,#50522,#50523,#50524,#50525,#50526,#50527,#50528,
#50529,#50530,#50531,#50532,#50533,#50534,#50535,#50536,#50537,#50538,#50539,
#50540,#50541,#50542,#50543,#50544,#50545,#50546,#50547,#50548,#50549,#50550,
#50551,#50552,#50553,#50554,#50555,#50556,#50557,#50558,#50559),
 .UNSPECIFIED.,.F.,.F.,(4,3,3,3,3,3,3,3,3,3,3,3,3,3,3,3,3,3,3,3,3,3,3,3,
3,3,3,3,3,3,3,3,3,3,3,3,3,3,3,3,3,4),(43.0671358448511,43.1654506943593,
43.263714257863,43.3619560390805,43.4602055127591,43.5585579544468,43.6569637991359,
43.755540573341,43.8296906333064,43.9282887583115,44.0267465410897,44.126969108862,
44.2252486665916,44.3234952456664,44.4217383287064,44.5234355173468,44.6218199307671,
44.7251735070177,44.8285270832683,44.9271252082715,45.0255829910477,45.1258055588205,
45.2240851165482,45.3223316956211,45.4205747786592,45.5222719673019,45.6206563807203,
45.7240099569752,45.8273635332301,45.9259616582337,46.0244194410103,46.124642008783,
46.222921566511,46.3211681455842,46.4194112286227,46.521108417265,46.6194928306837,
46.7228464069379,46.826199983192,46.9466622822371,47.0654828012677,47.1238896269617),
 .UNSPECIFIED.);
#472=B_SPLINE_CURVE_WITH_KNOTS('',3,(#50560,#50561,#50562,#50563,#50564,
#50565),.UNSPECIFIED.,.F.,.F.,(4,1,1,4),(47.123889803847,47.8250364331539,
48.8238728831158,49.3495871973939),.UNSPECIFIED.);
#473=B_SPLINE_CURVE_WITH_KNOTS('',3,(#50567,#50568,#50569,#50570,#50571,
#50572),.UNSPECIFIED.,.F.,.F.,(4,1,1,4),(47.1238901027736,47.3602297006343,
48.3590661505962,49.3496771194667),.UNSPECIFIED.);
#474=B_SPLINE_CURVE_WITH_KNOTS('',3,(#50573,#50574,#50575,#50576,#50577,
#50578,#50579,#50580,#50581,#50582,#50583,#50584,#50585,#50586,#50587,#50588,
#50589,#50590,#50591,#50592,#50593,#50594,#50595,#50596,#50597,#50598,#50599,
#50600,#50601,#50602,#50603,#50604,#50605,#50606,#50607,#50608,#50609,#50610,
#50611,#50612,#50613,#50614,#50615,#50616,#50617,#50618,#50619,#50620,#50621,
#50622,#50623,#50624,#50625,#50626,#50627,#50628,#50629,#50630,#50631,#50632,
#50633,#50634,#50635,#50636,#50637,#50638,#50639,#50640,#50641,#50642,#50643,
#50644,#50645,#50646,#50647,#50648,#50649,#50650,#50651,#50652,#50653,#50654,
#50655,#50656,#50657,#50658,#50659,#50660,#50661,#50662,#50663,#50664,#50665,
#50666,#50667,#50668,#50669,#50670,#50671,#50672,#50673,#50674,#50675,#50676,
#50677,#50678,#50679,#50680,#50681,#50682,#50683,#50684,#50685,#50686,#50687,
#50688,#50689,#50690,#50691,#50692,#50693,#50694,#50695,#50696),
 .UNSPECIFIED.,.F.,.F.,(4,3,3,3,3,3,3,3,3,3,3,3,3,3,3,3,3,3,3,3,3,3,3,3,
3,3,3,3,3,3,3,3,3,3,3,3,3,3,3,3,3,4),(43.0660207895399,43.1644088973725,
43.2646463990797,43.3648839007868,43.4634820258002,43.5619398085866,43.6621623763569,
43.7604419340951,43.8586885131787,43.9569315962275,44.0586287848578,44.157013198287,
44.2603667745178,44.3637203507487,44.4623184757498,44.5607762585239,44.6609988262972,
44.7592783840226,44.8575249630933,44.955768046129,45.0574652347744,45.1558496481904,
45.2592032244505,45.3625568007106,45.4611549257132,45.5596127084887,45.6598352762616,
45.7581148339886,45.8563614130607,45.9546044960983,46.0563016847418,46.1546860981594,
46.2580396744159,46.3613932506724,46.4587199838046,46.5559210250953,46.6530274701202,
46.750070296518,46.8471124553623,46.9441490048067,47.0412721236587,47.123889803847),
 .UNSPECIFIED.);
#475=B_SPLINE_CURVE_WITH_KNOTS('',3,(#50702,#50703,#50704,#50705,#50706,
#50707,#50708,#50709,#50710,#50711,#50712,#50713,#50714,#50715,#50716,#50717,
#50718,#50719,#50720,#50721,#50722,#50723,#50724,#50725,#50726,#50727,#50728,
#50729,#50730,#50731,#50732,#50733,#50734,#50735,#50736,#50737,#50738,#50739,
#50740,#50741,#50742,#50743,#50744,#50745,#50746,#50747,#50748,#50749,#50750,
#50751,#50752,#50753,#50754,#50755,#50756,#50757,#50758,#50759,#50760,#50761,
#50762,#50763,#50764,#50765,#50766,#50767,#50768,#50769,#50770,#50771,#50772,
#50773,#50774,#50775,#50776,#50777,#50778,#50779,#50780,#50781,#50782,#50783,
#50784,#50785,#50786,#50787,#50788,#50789,#50790,#50791,#50792,#50793,#50794,
#50795,#50796,#50797,#50798,#50799,#50800,#50801,#50802,#50803,#50804,#50805,
#50806,#50807,#50808,#50809,#50810,#50811,#50812,#50813,#50814,#50815,#50816,
#50817,#50818,#50819,#50820,#50821,#50822,#50823,#50824,#50825,#50826,#50827,
#50828),.UNSPECIFIED.,.F.,.F.,(4,3,3,3,3,3,3,3,3,3,3,3,3,3,3,3,3,3,3,3,
3,3,3,3,3,3,3,3,3,3,3,3,3,3,3,3,3,3,3,3,3,3,4),(36.7830721323901,36.8378354835733,
36.9364336084865,37.034891391171,37.1351139589666,37.2333935165987,37.3316400955749,
37.4298831785151,37.5315803672701,37.629964780589,37.7333183570621,37.8366719335352,
37.9352700586078,38.0337278414543,38.1339504092097,38.2322299670095,38.3304765461551,
38.4287196292662,38.5304168178239,38.6288012313158,38.7321548074064,38.835508383497,
38.9341065084864,39.0325642912488,39.1327868590251,39.2310664167388,39.3293129957978,
39.4275560788219,39.5292532674811,39.6276376808858,39.7309912571723,39.8343448334589,
39.9329429584521,40.0314007412181,40.1316233089935,40.2299028667104,40.3281494457725,
40.4263925287994,40.5280897174548,40.6264741308618,40.7298277071413,40.8331812834208,
40.8407044966674),.UNSPECIFIED.);
#476=B_SPLINE_CURVE_WITH_KNOTS('',3,(#50829,#50830,#50831,#50832,#50833,
#50834,#50835,#50836,#50837,#50838,#50839,#50840,#50841,#50842,#50843,#50844,
#50845,#50846,#50847,#50848,#50849,#50850,#50851,#50852,#50853,#50854,#50855,
#50856,#50857,#50858,#50859,#50860,#50861,#50862,#50863,#50864,#50865,#50866,
#50867,#50868,#50869,#50870,#50871,#50872,#50873,#50874,#50875,#50876,#50877,
#50878,#50879,#50880,#50881,#50882,#50883,#50884,#50885,#50886,#50887,#50888,
#50889,#50890,#50891,#50892,#50893,#50894,#50895,#50896,#50897,#50898),
 .UNSPECIFIED.,.F.,.F.,(4,3,3,3,3,3,3,3,3,3,3,3,3,3,3,3,3,3,3,3,3,3,3,4),
(40.8407044969197,40.93917053872,41.0374964280042,41.1368115911765,41.2349607512895,
41.3330774110131,41.4311912274065,41.5313978539005,41.6296531901077,41.7308354617452,
41.8320177333826,41.9306158583837,42.029073641158,42.1292962089313,42.2275757666567,
42.3258223457274,42.4240654287631,42.5257626174084,42.6241470308245,42.7275006070845,
42.8308541833445,42.9294559188132,43.0279051778277,43.0671358448511),
 .UNSPECIFIED.);
#477=B_SPLINE_CURVE_WITH_KNOTS('',3,(#50900,#50901,#50902,#50903,#50904,
#50905,#50906,#50907,#50908,#50909,#50910,#50911,#50912,#50913,#50914,#50915,
#50916,#50917,#50918,#50919,#50920,#50921,#50922,#50923,#50924,#50925,#50926,
#50927,#50928,#50929,#50930,#50931,#50932,#50933,#50934,#50935,#50936,#50937,
#50938,#50939,#50940,#50941,#50942,#50943,#50944,#50945,#50946,#50947,#50948,
#50949,#50950,#50951,#50952,#50953,#50954,#50955,#50956,#50957,#50958,#50959,
#50960,#50961,#50962,#50963,#50964,#50965,#50966,#50967,#50968,#50969),
 .UNSPECIFIED.,.F.,.F.,(4,3,3,3,3,3,3,3,3,3,3,3,3,3,3,3,3,3,3,3,3,3,3,4),
(40.8407044966674,40.942531041993,41.0487010317105,41.1508691915792,41.2531658485542,
41.3556785603229,41.3672110008631,41.4658091258526,41.5642669086151,41.6644894763913,
41.7627690341051,41.8610156131642,41.9592586961886,42.0609558848477,42.1593402982525,
42.2626938745387,42.3660474508249,42.46462340533,42.5630692109006,42.6614145831978,
42.7625661347833,42.8608128972949,42.9634168434174,43.0660207895399),
 .UNSPECIFIED.);
#478=B_SPLINE_CURVE_WITH_KNOTS('',3,(#50970,#50971,#50972,#50973,#50974,
#50975,#50976,#50977),.UNSPECIFIED.,.F.,.F.,(4,1,1,1,1,4),(36.7838197976209,
37.3718652010156,38.3707016509774,39.3695381009393,40.3683745509012,40.8407024149681),
 .UNSPECIFIED.);
#479=B_SPLINE_CURVE_WITH_KNOTS('',3,(#50983,#50984,#50985,#50986,#50987,
#50988,#50989,#50990,#50991,#50992,#50993,#50994,#50995,#50996,#50997,#50998,
#50999,#51000,#51001,#51002,#51003,#51004,#51005,#51006,#51007,#51008,#51009,
#51010,#51011,#51012,#51013,#51014,#51015,#51016,#51017,#51018,#51019,#51020,
#51021,#51022,#51023,#51024,#51025,#51026,#51027,#51028,#51029,#51030,#51031,
#51032,#51033,#51034,#51035,#51036,#51037,#51038,#51039,#51040,#51041,#51042,
#51043,#51044,#51045,#51046,#51047,#51048,#51049,#51050,#51051,#51052,#51053,
#51054,#51055,#51056,#51057,#51058,#51059,#51060,#51061,#51062,#51063,#51064,
#51065,#51066,#51067,#51068,#51069,#51070,#51071,#51072,#51073,#51074,#51075,
#51076,#51077,#51078,#51079,#51080,#51081,#51082,#51083,#51084,#51085,#51086,
#51087,#51088,#51089,#51090,#51091,#51092,#51093,#51094,#51095,#51096,#51097,
#51098,#51099,#51100,#51101,#51102,#51103,#51104,#51105,#51106,#51107,#51108,
#51109),.UNSPECIFIED.,.F.,.F.,(4,3,3,3,3,3,3,3,3,3,3,3,3,3,3,3,3,3,3,3,
3,3,3,3,3,3,3,3,3,3,3,3,3,3,3,3,3,3,3,3,3,3,4),(30.499739219623,30.5981024448967,
30.696525650912,30.7951123611512,30.844816783802,30.9434149029152,31.041872679698,
31.1420952489563,31.2403748004794,31.3386213732825,31.4368644499935,31.5385616459361,
31.6369460529487,31.7402996433563,31.8436532337639,31.9422513619745,32.0407091479983,
32.1409317149643,32.2392112760146,32.3374578584309,32.4357009448286,32.5373981295529,
32.6357825463377,32.7391361150317,32.8424896837258,32.9410878085145,33.0395455910813,
33.1397681589071,33.2380477164403,33.3362942953245,33.4345373781801,33.536234567057,
33.6346189803103,33.737972556999,33.8413261336877,33.9390973941501,34.0367388270535,
34.1342810926874,34.2317547370029,34.3292101035722,34.4266554953253,34.5241539309012,
34.5575191894878),.UNSPECIFIED.);
#480=B_SPLINE_CURVE_WITH_KNOTS('',3,(#51110,#51111,#51112,#51113,#51114,
#51115,#51116,#51117,#51118,#51119,#51120,#51121,#51122,#51123,#51124,#51125,
#51126,#51127,#51128,#51129,#51130,#51131,#51132,#51133,#51134,#51135,#51136,
#51137,#51138,#51139,#51140,#51141,#51142,#51143,#51144,#51145,#51146,#51147,
#51148,#51149,#51150,#51151,#51152,#51153,#51154,#51155,#51156,#51157,#51158,
#51159,#51160,#51161,#51162,#51163,#51164,#51165,#51166,#51167,#51168,#51169,
#51170,#51171,#51172,#51173,#51174,#51175,#51176,#51177,#51178,#51179),
 .UNSPECIFIED.,.F.,.F.,(4,3,3,3,3,3,3,3,3,3,3,3,3,3,3,3,3,3,3,3,3,3,3,4),
(34.5575191897594,34.6782345503606,34.8009387396023,34.8401625836495,34.9387607091287,
35.0372184923872,35.1374410600402,35.2357206182622,35.3339671978328,35.4322102813714,
35.5339074694314,35.6322918833521,35.7356454584817,35.8389990336114,35.9376008413508,
36.0360613066033,36.1344037647036,36.2326817408433,36.3309247589448,36.4291623016121,
36.5274785677211,36.6258371036476,36.7243383500819,36.7830721323901),
 .UNSPECIFIED.);
#481=B_SPLINE_CURVE_WITH_KNOTS('',3,(#51181,#51182,#51183,#51184,#51185,
#51186),.UNSPECIFIED.,.F.,.F.,(4,1,1,4),(34.5575241472562,35.3741923010918,
36.3730287510537,36.7838197976209),.UNSPECIFIED.);
#482=B_SPLINE_CURVE_WITH_KNOTS('',3,(#51187,#51188,#51189,#51190,#51191,
#51192,#51193,#51194,#51195,#51196,#51197,#51198,#51199,#51200,#51201,#51202,
#51203,#51204,#51205,#51206,#51207,#51208,#51209,#51210,#51211,#51212,#51213,
#51214,#51215,#51216,#51217,#51218,#51219,#51220,#51221,#51222,#51223,#51224,
#51225,#51226,#51227,#51228,#51229,#51230,#51231,#51232,#51233,#51234,#51235,
#51236,#51237,#51238,#51239,#51240,#51241,#51242,#51243,#51244,#51245,#51246,
#51247,#51248,#51249,#51250,#51251,#51252,#51253,#51254,#51255,#51256,#51257,
#51258,#51259,#51260,#51261,#51262,#51263,#51264,#51265,#51266,#51267,#51268,
#51269,#51270,#51271,#51272,#51273,#51274,#51275,#51276,#51277,#51278,#51279,
#51280,#51281,#51282,#51283,#51284,#51285,#51286,#51287,#51288,#51289,#51290,
#51291,#51292,#51293,#51294,#51295,#51296,#51297,#51298,#51299,#51300,#51301,
#51302,#51303,#51304,#51305,#51306,#51307,#51308,#51309,#51310),
 .UNSPECIFIED.,.F.,.F.,(4,3,3,3,3,3,3,3,3,3,3,3,3,3,3,3,3,3,3,3,3,3,3,3,
3,3,3,3,3,3,3,3,3,3,3,3,3,3,3,3,3,4),(30.5006744564005,30.5991052602797,
30.6974320559243,30.7957024047894,30.8939458184504,30.9921917748654,31.0905375599031,
31.1889321215594,31.2875030626886,31.3788465012443,31.4774446472214,31.5759024512158,
31.6761250137146,31.7744045931048,31.8726511939587,31.9708942988676,32.0725914619522,
32.170975897242,32.2743294242241,32.3776829512062,32.4762810765974,32.5747388598281,
32.6749614274956,32.7732409858386,32.8714875655859,32.9697306493566,33.0714278373095,
33.1698122515998,33.2731658263839,33.3765194011681,33.4751175203064,33.5735752971148,
33.6737978663667,33.7720774179164,33.8703239907463,33.9685670674843,34.0702642633957,
34.1686486704357,34.2720022607828,34.3753558511299,34.52385598093,34.5575191894878),
 .UNSPECIFIED.);
#483=B_SPLINE_CURVE_WITH_KNOTS('',3,(#51316,#51317,#51318,#51319,#51320,
#51321,#51322,#51323),.UNSPECIFIED.,.F.,.F.,(4,1,1,1,1,4),(24.2176478200484,
24.8517980840308,25.8506345339927,26.8494709839545,27.8483074339164,28.2743284148063),
 .UNSPECIFIED.);
#484=B_SPLINE_CURVE_WITH_KNOTS('',3,(#51324,#51325,#51326,#51327,#51328,
#51329,#51330,#51331,#51332,#51333,#51334,#51335,#51336,#51337,#51338,#51339,
#51340,#51341,#51342,#51343,#51344,#51345,#51346,#51347,#51348,#51349,#51350,
#51351,#51352,#51353,#51354,#51355,#51356,#51357,#51358,#51359,#51360,#51361,
#51362,#51363,#51364,#51365,#51366,#51367,#51368,#51369,#51370,#51371,#51372,
#51373,#51374,#51375,#51376,#51377,#51378,#51379,#51380,#51381,#51382,#51383,
#51384,#51385,#51386,#51387,#51388,#51389,#51390,#51391,#51392,#51393),
 .UNSPECIFIED.,.F.,.F.,(4,3,3,3,3,3,3,3,3,3,3,3,3,3,3,3,3,3,3,3,3,3,3,4),
(28.2743338823082,28.3746245106389,28.4749734038845,28.5754886320393,28.6760922702991,
28.7769068624285,28.8471438838783,28.9457420299505,29.044199834041,29.1444223965159,
29.2427019760043,29.3409485769571,29.4391916819651,29.5408888449339,29.6392732803231,
29.7426268070816,29.8459803338402,29.9445606477207,30.0430096057647,30.1413569295324,
30.2396381186448,30.3378792535309,30.4361386871605,30.499739219623),
 .UNSPECIFIED.);
#485=B_SPLINE_CURVE_WITH_KNOTS('',3,(#51395,#51396,#51397,#51398,#51399,
#51400,#51401,#51402,#51403,#51404,#51405,#51406,#51407,#51408,#51409,#51410,
#51411,#51412,#51413,#51414,#51415,#51416,#51417,#51418,#51419,#51420,#51421,
#51422,#51423,#51424,#51425,#51426,#51427,#51428,#51429,#51430,#51431,#51432,
#51433,#51434,#51435,#51436,#51437,#51438,#51439,#51440,#51441,#51442,#51443,
#51444,#51445,#51446,#51447,#51448,#51449,#51450,#51451,#51452,#51453,#51454,
#51455,#51456,#51457,#51458,#51459,#51460,#51461,#51462,#51463,#51464),
 .UNSPECIFIED.,.F.,.F.,(4,3,3,3,3,3,3,3,3,3,3,3,3,3,3,3,3,3,3,3,3,3,3,4),
(28.2743338823082,28.3823371513587,28.480935409995,28.5793933278136,28.679615862002,
28.7778955572416,28.8761422744467,28.9743854960547,29.0760825223712,29.1744670740333,
29.277820337677,29.3811736013206,29.479771742719,29.5782295425603,29.6784521061506,
29.7767316824742,29.8749782806757,29.9732213833518,30.0749185503344,30.1733029844702,
30.2766565178763,30.3800100512824,30.4786103666909,30.5006744564005),
 .UNSPECIFIED.);
#486=B_SPLINE_CURVE_WITH_KNOTS('',3,(#51465,#51466,#51467,#51468,#51469,
#51470,#51471,#51472,#51473,#51474,#51475,#51476,#51477,#51478,#51479,#51480,
#51481,#51482,#51483,#51484,#51485,#51486,#51487,#51488,#51489,#51490,#51491,
#51492,#51493,#51494,#51495,#51496,#51497,#51498,#51499,#51500,#51501,#51502,
#51503,#51504,#51505,#51506,#51507,#51508,#51509,#51510,#51511,#51512,#51513,
#51514,#51515,#51516,#51517,#51518,#51519,#51520,#51521,#51522,#51523,#51524,
#51525,#51526,#51527,#51528,#51529,#51530,#51531,#51532,#51533,#51534,#51535,
#51536,#51537,#51538,#51539,#51540,#51541,#51542,#51543,#51544,#51545,#51546,
#51547,#51548,#51549,#51550,#51551,#51552,#51553,#51554,#51555,#51556,#51557,
#51558,#51559,#51560,#51561,#51562,#51563,#51564,#51565,#51566,#51567,#51568,
#51569,#51570,#51571,#51572,#51573,#51574,#51575,#51576,#51577,#51578,#51579,
#51580,#51581,#51582,#51583,#51584,#51585,#51586,#51587,#51588,#51589,#51590,
#51591),.UNSPECIFIED.,.F.,.F.,(4,3,3,3,3,3,3,3,3,3,3,3,3,3,3,3,3,3,3,3,
3,3,3,3,3,3,3,3,3,3,3,3,3,3,3,3,3,3,3,3,3,3,4),(24.2164091248765,24.3149891714194,
24.3869913515112,24.4855869806887,24.584042229485,24.6842654259835,24.7825423743751,
24.8807863216562,24.9790267538739,25.0807270157737,25.1791087577961,25.2824682796346,
25.3858278014731,25.484426744909,25.5828853535715,25.6831077158044,25.781388111632,
25.8796355315209,25.9778794569755,26.0795756555903,26.1779609067728,26.2813125791038,
26.3846642514349,26.4832625887837,26.5817205899964,26.6819431039214,26.7802228935229,
26.8784697089924,26.9767130326531,27.078409949839,27.1767946120345,27.2801476567156,
27.3835007013968,27.4808124357131,27.5800026165089,27.6770619123618,27.7740624152157,
27.8710350591815,27.971859764906,28.0689211638456,28.1660361055543,28.2632831538734,
28.2743338820794),.UNSPECIFIED.);
#487=B_SPLINE_CURVE_WITH_KNOTS('',3,(#51597,#51598,#51599,#51600,#51601,
#51602),.UNSPECIFIED.,.F.,.F.,(4,1,1,4),(15.707963267949,16.3962997518162,
17.3951362017781,17.9335273566036),.UNSPECIFIED.);
#488=B_SPLINE_CURVE_WITH_KNOTS('',3,(#51604,#51605,#51606,#51607,#51608),
 .UNSPECIFIED.,.F.,.F.,(4,1,4),(14.3986268518925,15.3974633018543,15.707963267949),
 .UNSPECIFIED.);
#489=B_SPLINE_CURVE_WITH_KNOTS('',3,(#51612,#51613,#51614,#51615,#51616,
#51617,#51618,#51619,#51620,#51621,#51622,#51623,#51624,#51625,#51626,#51627,
#51628,#51629,#51630,#51631,#51632,#51633,#51634,#51635,#51636,#51637,#51638,
#51639,#51640,#51641,#51642,#51643,#51644,#51645,#51646,#51647,#51648,#51649,
#51650,#51651,#51652,#51653,#51654,#51655,#51656,#51657,#51658,#51659,#51660,
#51661,#51662,#51663,#51664,#51665,#51666,#51667,#51668,#51669),
 .UNSPECIFIED.,.F.,.F.,(4,3,3,3,3,3,3,3,3,3,3,3,3,3,3,3,3,3,3,4),(13.8757070305518,
13.9742335824856,14.0726198317922,14.1714715508697,14.2696802764454,14.3678558944916,
14.4660279816071,14.5653793823083,14.6636893819281,14.7635614831701,14.8634335844121,
14.9606976623845,15.0578044029831,15.1548229005499,15.2517842045426,15.3487192918042,
15.4457083561665,15.542724156859,15.6398692496992,15.707963267949),
 .UNSPECIFIED.);
#490=B_SPLINE_CURVE_WITH_KNOTS('',3,(#51670,#51671,#51672,#51673,#51674,
#51675,#51676),.UNSPECIFIED.,.F.,.F.,(4,1,1,1,4),(15.707963267949,15.8622700343739,
16.8611064843358,17.8599429342977,17.9342415884722),.UNSPECIFIED.);
#491=B_SPLINE_CURVE_WITH_KNOTS('',3,(#51682,#51683,#51684,#51685,#51686,
#51687,#51688,#51689),.UNSPECIFIED.,.F.,.F.,(4,1,1,1,1,4),(181.295997133577,
181.669120728045,182.667957178007,183.666793627969,184.665630077931,185.353966561798),
 .UNSPECIFIED.);
#492=B_SPLINE_CURVE_WITH_KNOTS('',3,(#51691,#51692,#51693,#51694,#51695),
 .UNSPECIFIED.,.F.,.F.,(4,1,4),(185.353966561798,185.664466527893,186.663302977854),
 .UNSPECIFIED.);
#493=B_SPLINE_CURVE_WITH_KNOTS('',3,(#51699,#51700,#51701,#51702,#51703,
#51704,#51705,#51706,#51707,#51708,#51709,#51710,#51711,#51712,#51713,#51714,
#51715,#51716,#51717,#51718,#51719,#51720,#51721,#51722,#51723,#51724,#51725,
#51726,#51727,#51728,#51729,#51730,#51731,#51732,#51733,#51734,#51735,#51736,
#51737,#51738,#51739,#51740,#51741,#51742,#51743,#51744,#51745,#51746,#51747,
#51748,#51749,#51750,#51751,#51752,#51753,#51754,#51755,#51756),
 .UNSPECIFIED.,.F.,.F.,(4,3,3,3,3,3,3,3,3,3,3,3,3,3,3,3,3,3,3,4),(185.353966561798,
185.451129857721,185.548173538225,185.645152135629,185.742096642157,185.839038005082,
185.936068670734,186.033145886574,186.130383559583,186.198496245335,186.297011743078,
186.39538923924,186.494243434233,186.592449062934,186.690623713446,186.78879696123,
186.88815342072,186.986469795236,187.086346297213,187.186222799189),
 .UNSPECIFIED.);
#494=B_SPLINE_CURVE_WITH_KNOTS('',3,(#51757,#51758,#51759,#51760,#51761,
#51762,#51763,#51764),.UNSPECIFIED.,.F.,.F.,(4,1,1,1,1,4),(181.2971675537,
182.203150445487,183.201986895449,184.200823345411,185.199659795373,185.353966561798),
 .UNSPECIFIED.);
#495=B_SPLINE_CURVE_WITH_KNOTS('',3,(#51770,#51771,#51772,#51773,#51774,
#51775,#51776,#51777,#51778,#51779,#51780,#51781,#51782,#51783,#51784,#51785,
#51786,#51787,#51788,#51789,#51790,#51791,#51792,#51793,#51794,#51795,#51796,
#51797,#51798,#51799,#51800,#51801,#51802,#51803,#51804,#51805,#51806,#51807,
#51808,#51809,#51810,#51811,#51812,#51813,#51814,#51815,#51816,#51817,#51818,
#51819,#51820,#51821,#51822,#51823,#51824,#51825,#51826,#51827,#51828,#51829,
#51830,#51831,#51832,#51833,#51834,#51835,#51836,#51837,#51838,#51839,#51840,
#51841,#51842,#51843,#51844,#51845,#51846,#51847,#51848,#51849,#51850,#51851,
#51852,#51853,#51854,#51855,#51856,#51857,#51858,#51859,#51860,#51861,#51862,
#51863,#51864,#51865,#51866,#51867,#51868,#51869,#51870,#51871,#51872,#51873,
#51874,#51875,#51876,#51877,#51878,#51879,#51880,#51881,#51882,#51883,#51884,
#51885,#51886,#51887,#51888,#51889,#51890,#51891,#51892,#51893),
 .UNSPECIFIED.,.F.,.F.,(4,3,3,3,3,3,3,3,3,3,3,3,3,3,3,3,3,3,3,3,3,3,3,3,
3,3,3,3,3,3,3,3,3,3,3,3,3,3,3,3,3,4),(175.013888660471,175.112152321306,
175.210394808164,175.308645594357,175.406999706945,175.50540776602,175.6039861128,
175.676102028274,175.774697485907,175.873152598171,175.973375833179,176.071652731782,
176.169896661679,176.268137108901,176.369837451234,176.468219288705,176.57157888347,
176.674938478236,176.77353909221,176.871999348327,176.972221295811,177.070503271432,
177.168752242674,177.266997689187,177.36869199894,177.467078681016,177.570426804607,
177.673774928198,177.772377764499,177.870840302866,177.971061687278,178.069346073991,
178.167597498754,178.265845437704,178.367536922818,178.465926167544,178.569268772851,
178.672611378159,178.782250111505,178.891545462336,179.000249339659,179.070781030153),
 .UNSPECIFIED.);
#496=B_SPLINE_CURVE_WITH_KNOTS('',3,(#51894,#51895,#51896,#51897,#51898,
#51899),.UNSPECIFIED.,.F.,.F.,(4,1,1,4),(179.070781254618,179.671447828121,
180.670284278083,181.295997133577),.UNSPECIFIED.);
#497=B_SPLINE_CURVE_WITH_KNOTS('',3,(#51901,#51902,#51903,#51904,#51905,
#51906,#51907),.UNSPECIFIED.,.F.,.F.,(4,1,1,1,4),(179.070781254618,179.206641095602,
180.205477545564,181.204313995525,181.2971675537),.UNSPECIFIED.);
#498=B_SPLINE_CURVE_WITH_KNOTS('',3,(#51908,#51909,#51910,#51911,#51912,
#51913,#51914,#51915),.UNSPECIFIED.,.F.,.F.,(4,1,1,1,1,4),(175.012544821303,
175.211295295754,176.210131745716,177.208968195678,178.20780464564,179.070781254618),
 .UNSPECIFIED.);
#499=B_SPLINE_CURVE_WITH_KNOTS('',3,(#51921,#51922,#51923,#51924,#51925,
#51926,#51927,#51928,#51929,#51930,#51931,#51932,#51933,#51934,#51935,#51936,
#51937,#51938,#51939,#51940,#51941,#51942,#51943,#51944,#51945,#51946,#51947,
#51948,#51949,#51950,#51951,#51952,#51953,#51954,#51955,#51956,#51957,#51958,
#51959,#51960,#51961,#51962,#51963,#51964,#51965,#51966,#51967,#51968,#51969,
#51970,#51971,#51972,#51973,#51974,#51975,#51976,#51977,#51978,#51979,#51980,
#51981,#51982,#51983,#51984,#51985,#51986,#51987,#51988,#51989,#51990,#51991,
#51992,#51993,#51994,#51995,#51996,#51997,#51998,#51999,#52000,#52001,#52002,
#52003,#52004,#52005,#52006,#52007,#52008,#52009,#52010,#52011,#52012,#52013,
#52014,#52015,#52016,#52017,#52018,#52019,#52020,#52021,#52022,#52023,#52024,
#52025,#52026,#52027,#52028,#52029,#52030,#52031,#52032,#52033,#52034,#52035,
#52036,#52037,#52038,#52039,#52040,#52041,#52042,#52043,#52044),
 .UNSPECIFIED.,.F.,.F.,(4,3,3,3,3,3,3,3,3,3,3,3,3,3,3,3,3,3,3,3,3,3,3,3,
3,3,3,3,3,3,3,3,3,3,3,3,3,3,3,3,3,4),(168.730499549008,168.829027791897,
168.927431101866,169.025741410082,169.124002504523,169.222243885976,169.320495028123,
169.41885037296,169.517260979166,169.615840378079,169.683083328503,169.781681404542,
169.880139138361,169.980361718374,170.078641227507,170.176887758226,170.27513079321,
170.376828039524,170.475212406123,170.578566092293,170.681919778464,170.780517924866,
170.878975728651,170.979198291123,171.077477868767,171.17572446731,171.273967569349,
171.375664734118,171.474049165187,171.577402696807,171.680756228426,171.779354490553,
171.877812411242,171.978034944635,172.076314641203,172.17456135916,172.272804580942,
172.374501605303,172.472886155702,172.576239417045,172.679592678388,172.787595947439),
 .UNSPECIFIED.);
#500=B_SPLINE_CURVE_WITH_KNOTS('',3,(#52045,#52046,#52047,#52048,#52049,
#52050,#52051,#52052,#52053,#52054,#52055,#52056,#52057,#52058,#52059,#52060,
#52061,#52062,#52063,#52064,#52065,#52066,#52067,#52068,#52069,#52070,#52071,
#52072,#52073,#52074,#52075,#52076,#52077,#52078,#52079,#52080,#52081,#52082,
#52083,#52084,#52085,#52086,#52087,#52088,#52089,#52090,#52091,#52092,#52093,
#52094,#52095,#52096,#52097,#52098,#52099,#52100,#52101,#52102,#52103,#52104,
#52105,#52106,#52107,#52108,#52109,#52110,#52111,#52112,#52113,#52114,#52115,
#52116,#52117),.UNSPECIFIED.,.F.,.F.,(4,3,3,3,3,3,3,3,3,3,3,3,3,3,3,3,3,
3,3,3,3,3,3,3,4),(172.787595947668,172.884841558603,172.984040004821,173.081071836984,
173.178059268517,173.275033212281,173.375882191298,173.472980624789,173.57014496826,
173.66745840562,173.67842912835,173.777027506535,173.875485539983,173.975708044774,
174.073987845308,174.172234663756,174.270477982445,174.372174881412,174.470559518906,
174.573912548609,174.677265578312,174.77584482842,174.874301068252,174.972645515065,
175.013888660471),.UNSPECIFIED.);
#501=B_SPLINE_CURVE_WITH_KNOTS('',3,(#52119,#52120,#52121,#52122,#52123,
#52124),.UNSPECIFIED.,.F.,.F.,(4,1,1,4),(172.787601414694,173.21362239583,
174.212458845792,175.012544821303),.UNSPECIFIED.);
#502=B_SPLINE_CURVE_WITH_KNOTS('',3,(#52125,#52126,#52127,#52128,#52129,
#52130,#52131,#52132,#52133,#52134,#52135,#52136,#52137,#52138,#52139,#52140,
#52141,#52142,#52143,#52144,#52145,#52146,#52147,#52148,#52149,#52150,#52151,
#52152,#52153,#52154,#52155,#52156,#52157,#52158,#52159,#52160,#52161,#52162,
#52163,#52164,#52165,#52166,#52167,#52168,#52169,#52170,#52171,#52172,#52173,
#52174,#52175,#52176,#52177,#52178,#52179,#52180,#52181,#52182,#52183,#52184,
#52185,#52186,#52187,#52188,#52189,#52190,#52191,#52192,#52193,#52194,#52195,
#52196,#52197,#52198,#52199,#52200,#52201,#52202,#52203,#52204,#52205,#52206,
#52207,#52208,#52209,#52210,#52211,#52212,#52213,#52214,#52215,#52216,#52217,
#52218,#52219,#52220,#52221,#52222,#52223,#52224,#52225,#52226,#52227,#52228,
#52229,#52230,#52231,#52232,#52233,#52234,#52235,#52236,#52237,#52238,#52239,
#52240,#52241,#52242,#52243,#52244,#52245,#52246,#52247,#52248),
 .UNSPECIFIED.,.F.,.F.,(4,3,3,3,3,3,3,3,3,3,3,3,3,3,3,3,3,3,3,3,3,3,3,3,
3,3,3,3,3,3,3,3,3,3,3,3,3,3,3,3,3,4),(168.73021510062,168.828460568105,
168.926805276369,169.025197909693,169.12376794625,169.218276595983,169.316874714607,
169.41533249101,169.515555060377,169.613834611791,169.712081184585,169.810324261387,
169.912021457527,170.01040586488,170.113759455413,170.217113045945,170.315711171923,
170.414168955615,170.514391523152,170.612671081648,170.710917661432,170.809160745125,
170.910857932821,171.009242346748,171.112595921327,171.215949495907,171.314547642568,
171.413005447104,171.513228009449,171.611507589026,171.709754189934,171.807997294764,
171.90969445754,172.008078892422,172.111432419146,172.214785945869,172.315617765325,
172.416285943672,172.516781875576,172.617176498836,172.717484580328,172.787595947439),
 .UNSPECIFIED.);
#503=B_SPLINE_CURVE_WITH_KNOTS('',3,(#52254,#52255,#52256,#52257,#52258,
#52259,#52260,#52261),.UNSPECIFIED.,.F.,.F.,(4,1,1,1,1,4),(162.446146734229,
162.691228178769,163.690064628731,164.688901078693,165.687737528655,166.504405683232),
 .UNSPECIFIED.);
#504=B_SPLINE_CURVE_WITH_KNOTS('',3,(#52262,#52263,#52264,#52265,#52266,
#52267,#52268,#52269,#52270,#52271,#52272,#52273,#52274,#52275,#52276,#52277,
#52278,#52279,#52280,#52281,#52282,#52283,#52284,#52285,#52286,#52287,#52288,
#52289,#52290,#52291,#52292,#52293,#52294,#52295,#52296,#52297,#52298,#52299,
#52300,#52301,#52302,#52303,#52304,#52305,#52306,#52307,#52308,#52309,#52310,
#52311,#52312,#52313,#52314,#52315,#52316,#52317,#52318,#52319,#52320,#52321,
#52322,#52323,#52324,#52325,#52326,#52327,#52328,#52329,#52330,#52331),
 .UNSPECIFIED.,.F.,.F.,(4,3,3,3,3,3,3,3,3,3,3,3,3,3,3,3,3,3,3,3,3,3,3,4),
(166.504410640259,166.652910770227,166.686573978617,166.785172097216,166.883629873594,
166.983852442967,167.082131994355,167.180378567125,167.278621643903,167.380318840072,
167.478703247402,167.58205683799,167.685410428579,167.784008554554,167.882466338243,
167.98268890578,168.080968464272,168.179215044053,168.277458127742,168.379155315442,
168.477539729364,168.580893303952,168.684246878541,168.730499549008),
 .UNSPECIFIED.);
#505=B_SPLINE_CURVE_WITH_KNOTS('',3,(#52333,#52334,#52335,#52336,#52337,
#52338,#52339,#52340,#52341,#52342,#52343,#52344,#52345,#52346,#52347,#52348,
#52349,#52350,#52351,#52352,#52353,#52354,#52355,#52356,#52357,#52358,#52359,
#52360,#52361,#52362,#52363,#52364,#52365,#52366,#52367,#52368,#52369,#52370,
#52371,#52372,#52373,#52374,#52375,#52376,#52377,#52378,#52379,#52380,#52381,
#52382,#52383,#52384,#52385,#52386,#52387,#52388,#52389,#52390,#52391,#52392,
#52393,#52394,#52395,#52396,#52397,#52398,#52399,#52400,#52401,#52402,#52403,
#52404,#52405),.UNSPECIFIED.,.F.,.F.,(4,3,3,3,3,3,3,3,3,3,3,3,3,3,3,3,3,
3,3,3,3,3,3,3,4),(166.504410640259,166.6019131263,166.699371433809,166.79681599036,
166.894277201724,166.991846173228,167.089478292237,167.187269535439,167.220603696059,
167.319201820915,167.417659603535,167.517882171346,167.616161728898,167.714408307788,
167.812651390637,167.914348579483,168.012732992698,168.116086569359,168.219440146021,
168.318036793094,168.421081369976,168.519419921282,168.617691702015,168.715928374415,
168.73021510062),.UNSPECIFIED.);
#506=B_SPLINE_CURVE_WITH_KNOTS('',3,(#52406,#52407,#52408,#52409,#52410,
#52411,#52412,#52413,#52414,#52415,#52416,#52417,#52418,#52419,#52420,#52421,
#52422,#52423,#52424,#52425,#52426,#52427,#52428,#52429,#52430,#52431,#52432,
#52433,#52434,#52435,#52436,#52437,#52438,#52439,#52440,#52441,#52442,#52443,
#52444,#52445,#52446,#52447,#52448,#52449,#52450,#52451,#52452,#52453,#52454,
#52455,#52456,#52457,#52458,#52459,#52460,#52461,#52462,#52463,#52464,#52465,
#52466,#52467,#52468,#52469,#52470,#52471,#52472,#52473,#52474,#52475,#52476,
#52477,#52478,#52479,#52480,#52481,#52482,#52483,#52484,#52485,#52486,#52487,
#52488,#52489,#52490,#52491,#52492,#52493,#52494,#52495,#52496,#52497,#52498,
#52499,#52500,#52501,#52502,#52503,#52504,#52505,#52506,#52507,#52508,#52509,
#52510,#52511,#52512,#52513,#52514,#52515,#52516,#52517,#52518,#52519,#52520,
#52521,#52522,#52523,#52524,#52525,#52526,#52527,#52528,#52529),
 .UNSPECIFIED.,.F.,.F.,(4,3,3,3,3,3,3,3,3,3,3,3,3,3,3,3,3,3,3,3,3,3,3,3,
3,3,3,3,3,3,3,3,3,3,3,3,3,3,3,3,3,4),(162.447662236975,162.545987533319,
162.644257027658,162.742500230488,162.840746619266,162.939093233869,163.03748920276,
163.136060860489,163.225257896212,163.323856021116,163.422313803793,163.522536371591,
163.620815929221,163.719062508197,163.817305591139,163.919002779898,164.017387193223,
164.120740769699,164.224094346174,164.322692471118,164.421150253833,164.521372821621,
164.619652379285,164.717898958294,164.816142041267,164.917839229985,165.016223643337,
165.119577219737,165.222930796136,165.321528921635,165.419986704909,165.520209272558,
165.618488830783,165.716735410353,165.814978493886,165.916675681939,166.015060095843,
166.11841367097,166.221767246097,166.34459987441,166.465474953157,166.504410639987),
 .UNSPECIFIED.);
#507=B_SPLINE_CURVE_WITH_KNOTS('',3,(#52535,#52536,#52537,#52538,#52539,
#52540,#52541,#52542,#52543,#52544,#52545,#52546,#52547,#52548,#52549,#52550,
#52551,#52552,#52553,#52554,#52555,#52556,#52557,#52558,#52559,#52560,#52561,
#52562,#52563,#52564,#52565,#52566,#52567,#52568,#52569,#52570,#52571,#52572,
#52573,#52574,#52575,#52576,#52577,#52578,#52579,#52580,#52581,#52582,#52583,
#52584,#52585,#52586,#52587,#52588,#52589,#52590,#52591,#52592,#52593,#52594,
#52595,#52596,#52597,#52598,#52599,#52600,#52601,#52602,#52603,#52604,#52605,
#52606,#52607,#52608,#52609,#52610,#52611,#52612,#52613,#52614,#52615,#52616,
#52617,#52618,#52619,#52620,#52621,#52622,#52623,#52624,#52625,#52626,#52627,
#52628,#52629,#52630,#52631,#52632,#52633,#52634,#52635,#52636,#52637,#52638,
#52639,#52640,#52641,#52642,#52643,#52644,#52645,#52646,#52647,#52648,#52649,
#52650,#52651,#52652,#52653,#52654,#52655,#52656,#52657,#52658,#52659,#52660,
#52661),.UNSPECIFIED.,.F.,.F.,(4,3,3,3,3,3,3,3,3,3,3,3,3,3,3,3,3,3,3,3,
3,3,3,3,3,3,3,3,3,3,3,3,3,3,3,3,3,3,3,3,3,3,4),(156.163987595307,156.262228639747,
156.360486901622,156.458853695073,156.557282451664,156.655872548919,156.698209478998,
156.796807604012,156.895265386799,156.995487954569,157.093767512308,157.192014091392,
157.29025717444,157.39195436307,157.490338776499,157.59369235273,157.69704592896,
157.795644053952,157.894101836717,157.994324404493,158.092603962209,158.190850541271,
158.289093624298,158.390790812954,158.489175226362,158.592528802642,158.695882378922,
158.794480503912,158.892938286675,158.993160854451,159.091440412165,159.189686991224,
159.287930074247,159.389627262907,159.488011676311,159.591365252598,159.694718828884,
159.797216560019,159.903218753284,160.005303397592,160.107256278837,160.209067828956,
160.22122533308),.UNSPECIFIED.);
#508=B_SPLINE_CURVE_WITH_KNOTS('',3,(#52662,#52663,#52664,#52665,#52666,
#52667),.UNSPECIFIED.,.F.,.F.,(4,1,1,4),(160.221227414878,160.693555278846,
161.692391728808,162.446146734229),.UNSPECIFIED.);
#509=B_SPLINE_CURVE_WITH_KNOTS('',3,(#52669,#52670,#52671,#52672,#52673,
#52674,#52675,#52676,#52677,#52678,#52679,#52680,#52681,#52682,#52683,#52684,
#52685,#52686,#52687,#52688,#52689,#52690,#52691,#52692,#52693,#52694,#52695,
#52696,#52697,#52698,#52699,#52700,#52701,#52702,#52703,#52704,#52705,#52706,
#52707,#52708,#52709,#52710,#52711,#52712,#52713,#52714,#52715,#52716,#52717,
#52718,#52719,#52720,#52721,#52722,#52723,#52724,#52725,#52726,#52727,#52728,
#52729,#52730,#52731,#52732,#52733,#52734,#52735,#52736,#52737,#52738,#52739,
#52740,#52741),.UNSPECIFIED.,.F.,.F.,(4,3,3,3,3,3,3,3,3,3,3,3,3,3,3,3,3,
3,3,3,3,3,3,3,4),(160.22122533308,160.228748546326,160.327346671318,160.425804454083,
160.526027021859,160.624306579575,160.722553158637,160.820796241665,160.92249343032,
161.020877843728,161.124231420008,161.227584996288,161.326183121278,161.424640904041,
161.524863471817,161.623143029531,161.72138960859,161.819632691614,161.921329880273,
162.019714293678,162.123067869964,162.22642144625,162.325027405982,162.423481500059,
162.447662236975),.UNSPECIFIED.);
#510=B_SPLINE_CURVE_WITH_KNOTS('',3,(#52742,#52743,#52744,#52745,#52746,
#52747,#52748,#52749,#52750,#52751,#52752,#52753,#52754,#52755,#52756,#52757,
#52758,#52759,#52760,#52761,#52762,#52763,#52764,#52765,#52766,#52767,#52768,
#52769,#52770,#52771,#52772,#52773,#52774,#52775,#52776,#52777,#52778,#52779,
#52780,#52781,#52782,#52783,#52784,#52785,#52786,#52787,#52788,#52789,#52790,
#52791,#52792,#52793,#52794,#52795,#52796,#52797,#52798,#52799,#52800,#52801,
#52802,#52803,#52804,#52805,#52806,#52807,#52808,#52809,#52810,#52811,#52812,
#52813,#52814,#52815,#52816,#52817,#52818,#52819,#52820,#52821,#52822,#52823,
#52824,#52825,#52826,#52827,#52828,#52829,#52830,#52831,#52832,#52833,#52834,
#52835,#52836,#52837,#52838,#52839,#52840,#52841,#52842,#52843,#52844,#52845,
#52846,#52847,#52848,#52849,#52850,#52851,#52852,#52853,#52854,#52855,#52856,
#52857,#52858,#52859,#52860,#52861,#52862,#52863,#52864,#52865),
 .UNSPECIFIED.,.F.,.F.,(4,3,3,3,3,3,3,3,3,3,3,3,3,3,3,3,3,3,3,3,3,3,3,3,
3,3,3,3,3,3,3,3,3,3,3,3,3,3,3,3,3,4),(156.163531931712,156.233402746479,
156.332000871484,156.430458654262,156.530681222035,156.628960779764,156.727207358839,
156.825450441879,156.927147630519,157.025532043939,157.12888562019,157.232239196441,
157.330837321443,157.429295104219,157.529517671992,157.627797229718,157.72604380879,
157.824286891828,157.925984080471,158.024368493889,158.127722070145,158.231075646402,
158.329673771403,158.428131554177,158.528354121951,158.626633679676,158.724880258747,
158.823123341783,158.924820530428,159.023204943844,159.126558520104,159.229912096364,
159.328378576654,159.426704810661,159.526019875932,159.624169149678,159.722285836342,
159.820399593048,159.920606027993,160.018861091251,160.120043212039,160.221225332828),
 .UNSPECIFIED.);
#511=B_SPLINE_CURVE_WITH_KNOTS('',3,(#52871,#52872,#52873,#52874,#52875,
#52876,#52877,#52878),.UNSPECIFIED.,.F.,.F.,(4,1,1,1,1,4),(149.881541704413,
150.705190779227,151.704027229189,152.702863679151,153.701700129113,153.938039726298),
 .UNSPECIFIED.);
#512=B_SPLINE_CURVE_WITH_KNOTS('',3,(#52879,#52880,#52881,#52882,#52883,
#52884,#52885,#52886,#52887,#52888,#52889,#52890,#52891,#52892,#52893,#52894,
#52895,#52896,#52897,#52898,#52899,#52900,#52901,#52902,#52903,#52904,#52905,
#52906,#52907,#52908,#52909,#52910,#52911,#52912,#52913,#52914,#52915,#52916,
#52917,#52918,#52919,#52920,#52921,#52922,#52923,#52924,#52925,#52926,#52927,
#52928,#52929,#52930,#52931,#52932,#52933,#52934,#52935,#52936,#52937,#52938,
#52939,#52940,#52941,#52942,#52943,#52944,#52945,#52946,#52947,#52948),
 .UNSPECIFIED.,.F.,.F.,(4,3,3,3,3,3,3,3,3,3,3,3,3,3,3,3,3,3,3,3,3,3,3,4),
(153.9380400259,154.035163898234,154.132222574363,154.229246955324,154.326267897773,
154.423381488606,154.520541056366,154.617870832504,154.700536579074,154.799134704076,
154.897592486852,154.997815054625,155.096094612352,155.194341191424,155.292584274461,
155.394281463105,155.492665876522,155.596019452779,155.699373029036,155.79797586222,
155.89641514303,155.9947593991,156.093038592392,156.163987595307),
 .UNSPECIFIED.);
#513=B_SPLINE_CURVE_WITH_KNOTS('',3,(#52950,#52951,#52952,#52953,#52954,
#52955,#52956,#52957,#52958,#52959,#52960,#52961,#52962,#52963,#52964,#52965,
#52966,#52967,#52968,#52969,#52970,#52971,#52972,#52973,#52974,#52975,#52976,
#52977,#52978,#52979,#52980,#52981,#52982,#52983,#52984,#52985,#52986,#52987,
#52988,#52989,#52990,#52991,#52992,#52993,#52994,#52995,#52996,#52997,#52998,
#52999,#53000,#53001,#53002,#53003,#53004,#53005,#53006,#53007,#53008,#53009,
#53010,#53011,#53012,#53013,#53014,#53015,#53016,#53017,#53018,#53019),
 .UNSPECIFIED.,.F.,.F.,(4,3,3,3,3,3,3,3,3,3,3,3,3,3,3,3,3,3,3,3,3,3,3,4),
(153.938040202766,154.056659980235,154.176963650991,154.235729846555,154.334327971559,
154.432785754335,154.533008322108,154.631287879836,154.729534458909,154.827777541948,
154.92947473059,155.027859144009,155.131212720263,155.234566296517,155.33316914801,
155.431630381046,155.529972651698,155.628250049481,155.726492098718,155.82472828193,
155.923038846793,156.021391522283,156.119876942737,156.163531931712),
 .UNSPECIFIED.);
#514=B_SPLINE_CURVE_WITH_KNOTS('',3,(#53020,#53021,#53022,#53023,#53024,
#53025,#53026,#53027),.UNSPECIFIED.,.F.,.F.,(4,1,1,1,1,4),(149.880018495728,
150.240384046707,151.239220496669,152.238056946631,153.236893396593,153.9380400259),
 .UNSPECIFIED.);
#515=B_SPLINE_CURVE_WITH_KNOTS('',3,(#53033,#53034,#53035,#53036,#53037,
#53038,#53039,#53040,#53041,#53042,#53043,#53044,#53045,#53046,#53047,#53048,
#53049,#53050,#53051,#53052,#53053,#53054,#53055,#53056,#53057,#53058,#53059,
#53060,#53061,#53062,#53063,#53064,#53065,#53066,#53067,#53068,#53069,#53070,
#53071,#53072,#53073,#53074,#53075,#53076,#53077,#53078,#53079,#53080,#53081,
#53082,#53083,#53084,#53085,#53086,#53087,#53088,#53089,#53090,#53091,#53092,
#53093,#53094,#53095,#53096,#53097,#53098,#53099,#53100,#53101,#53102,#53103,
#53104,#53105,#53106,#53107,#53108,#53109,#53110,#53111,#53112,#53113,#53114,
#53115,#53116,#53117,#53118,#53119,#53120,#53121,#53122,#53123,#53124,#53125,
#53126,#53127,#53128,#53129,#53130,#53131,#53132,#53133,#53134,#53135,#53136,
#53137,#53138,#53139,#53140,#53141,#53142,#53143,#53144,#53145,#53146,#53147,
#53148,#53149,#53150,#53151,#53152,#53153,#53154,#53155,#53156,#53157,#53158,
#53159),.UNSPECIFIED.,.F.,.F.,(4,3,3,3,3,3,3,3,3,3,3,3,3,3,3,3,3,3,3,3,
3,3,3,3,3,3,3,3,3,3,3,3,3,3,3,3,3,3,3,3,3,3,4),(143.597018511536,143.695621253918,
143.713335629494,143.811933754498,143.910391537274,144.010614105047,144.108893662775,
144.207140241849,144.305383324887,144.407080513529,144.505464926948,144.608818503202,
144.712172079456,144.81077020446,144.909227987236,145.009450555009,145.107730112737,
145.205976691811,145.304219774849,145.405916963491,145.50430137691,145.607654953164,
145.711008529418,145.809606654422,145.908064437198,146.008287004971,146.106566562699,
146.204813141772,146.303056224811,146.404753413453,146.503137826872,146.606491403125,
146.709844979379,146.807643480436,146.905302408374,147.002849316603,147.100335701354,
147.197792033696,147.295248746519,147.3927980835,147.490396206244,147.588155506493,
147.65485471872),.UNSPECIFIED.);
#516=B_SPLINE_CURVE_WITH_KNOTS('',3,(#53160,#53161,#53162,#53163,#53164,
#53165,#53166),.UNSPECIFIED.,.F.,.F.,(4,1,1,1,4),(147.65485471872,147.708681429341,
148.707517879303,149.706354329265,149.881541704413),.UNSPECIFIED.);
#517=B_SPLINE_CURVE_WITH_KNOTS('',3,(#53168,#53169,#53170,#53171,#53172,
#53173),.UNSPECIFIED.,.F.,.F.,(4,1,1,4),(147.65485471872,148.242711146784,
149.241547596746,149.880018495728),.UNSPECIFIED.);
#518=B_SPLINE_CURVE_WITH_KNOTS('',3,(#53174,#53175,#53176,#53177,#53178,
#53179,#53180,#53181,#53182,#53183,#53184,#53185,#53186,#53187,#53188,#53189,
#53190,#53191,#53192,#53193,#53194,#53195,#53196,#53197,#53198,#53199,#53200,
#53201,#53202,#53203,#53204,#53205,#53206,#53207,#53208,#53209,#53210,#53211,
#53212,#53213,#53214,#53215,#53216,#53217,#53218,#53219,#53220,#53221,#53222,
#53223,#53224,#53225,#53226,#53227,#53228,#53229,#53230,#53231,#53232,#53233,
#53234,#53235,#53236,#53237,#53238,#53239,#53240,#53241,#53242,#53243,#53244,
#53245,#53246,#53247,#53248,#53249,#53250,#53251,#53252,#53253,#53254,#53255,
#53256,#53257,#53258,#53259,#53260,#53261,#53262,#53263,#53264,#53265,#53266,
#53267,#53268,#53269,#53270,#53271,#53272,#53273,#53274,#53275,#53276,#53277,
#53278,#53279,#53280,#53281,#53282,#53283,#53284,#53285,#53286,#53287,#53288,
#53289,#53290,#53291,#53292,#53293,#53294,#53295,#53296,#53297),
 .UNSPECIFIED.,.F.,.F.,(4,3,3,3,3,3,3,3,3,3,3,3,3,3,3,3,3,3,3,3,3,3,3,3,
3,3,3,3,3,3,3,3,3,3,3,3,3,3,3,3,3,4),(143.597933925136,143.69619231975,
143.794433374417,143.892686561819,143.99104535005,144.089461531313,144.188044092565,
144.247365346936,144.34596347194,144.444421254716,144.544643822489,144.642923380217,
144.741169959291,144.839413042329,144.941110230972,145.03949464439,145.142848220644,
145.246201796898,145.344799921902,145.443257704679,145.543480272451,145.64175983018,
145.740006409253,145.838249492292,145.939946680934,146.038331094352,146.141684670606,
146.24503824686,146.343636371864,146.442094154641,146.542316722413,146.640596280141,
146.738842859215,146.837085942254,146.938783130896,147.037167544314,147.140521120568,
147.243874696822,147.352569174392,147.460952550046,147.568802109382,147.654854305399),
 .UNSPECIFIED.);
#519=B_SPLINE_CURVE_WITH_KNOTS('',3,(#53303,#53304,#53305,#53306,#53307,
#53308,#53309,#53310,#53311,#53312,#53313,#53314,#53315,#53316,#53317,#53318,
#53319,#53320,#53321,#53322,#53323,#53324,#53325,#53326,#53327,#53328,#53329,
#53330,#53331,#53332,#53333,#53334,#53335,#53336,#53337,#53338,#53339,#53340,
#53341,#53342,#53343,#53344,#53345,#53346,#53347,#53348,#53349,#53350,#53351,
#53352,#53353,#53354,#53355,#53356,#53357,#53358,#53359,#53360,#53361,#53362,
#53363,#53364,#53365,#53366,#53367,#53368,#53369,#53370,#53371,#53372,#53373,
#53374,#53375,#53376,#53377,#53378,#53379,#53380,#53381,#53382,#53383,#53384,
#53385,#53386,#53387,#53388,#53389,#53390,#53391,#53392,#53393,#53394,#53395,
#53396,#53397,#53398,#53399,#53400,#53401,#53402,#53403,#53404,#53405,#53406,
#53407,#53408,#53409,#53410,#53411,#53412,#53413,#53414,#53415,#53416,#53417,
#53418,#53419,#53420,#53421,#53422,#53423,#53424,#53425,#53426),
 .UNSPECIFIED.,.F.,.F.,(4,3,3,3,3,3,3,3,3,3,3,3,3,3,3,3,3,3,3,3,3,3,3,3,
3,3,3,3,3,3,3,3,3,3,3,3,3,3,3,3,3,4),(137.314044096691,137.415612304949,
137.51399694479,137.617156937256,137.720316929723,137.818915054726,137.917372837503,
138.017595405276,138.115874963004,138.214121542077,138.312364625116,138.414061813758,
138.512446227177,138.61579980343,138.719153379684,138.817751504688,138.916209287465,
139.016431855237,139.114711412965,139.212957992039,139.311201075077,139.412898263719,
139.511282677138,139.614636253392,139.717989829646,139.81658795465,139.915045737427,
140.015268305199,140.113547862927,140.211794442001,140.310037525039,140.411734713681,
140.5101191271,140.613472703354,140.716826279608,140.815569227393,140.914173010821,
141.012667061738,141.11108183093,141.209449097701,141.307822396311,141.371669411541),
 .UNSPECIFIED.);
#520=B_SPLINE_CURVE_WITH_KNOTS('',3,(#53427,#53428,#53429,#53430,#53431,
#53432,#53433,#53434,#53435,#53436,#53437,#53438,#53439,#53440,#53441,#53442,
#53443,#53444,#53445,#53446,#53447,#53448,#53449,#53450,#53451,#53452,#53453,
#53454,#53455,#53456,#53457,#53458,#53459,#53460,#53461,#53462,#53463,#53464,
#53465,#53466,#53467,#53468,#53469,#53470,#53471,#53472,#53473,#53474,#53475,
#53476,#53477,#53478,#53479,#53480,#53481,#53482,#53483,#53484,#53485,#53486,
#53487,#53488,#53489,#53490,#53491,#53492,#53493),.UNSPECIFIED.,.F.,.F.,
(4,3,3,3,3,3,3,3,3,3,3,3,3,3,3,3,3,3,3,3,3,3,4),(141.371669411768,141.485016004534,
141.600339367052,141.71566272957,141.814260854574,141.91271863735,142.012941205123,
142.111220762851,142.209467341925,142.307710424963,142.409407613605,142.507792027024,
142.611145603278,142.714499179532,142.813105314795,142.911543009964,143.009885026327,
143.108160960053,143.206400336867,143.304679404128,143.402973649661,143.501391759164,
143.597018511536),.UNSPECIFIED.);
#521=B_SPLINE_CURVE_WITH_KNOTS('',3,(#53495,#53496,#53497,#53498,#53499,
#53500,#53501,#53502,#53503,#53504,#53505,#53506,#53507,#53508,#53509,#53510,
#53511,#53512,#53513,#53514,#53515,#53516,#53517,#53518,#53519,#53520,#53521,
#53522,#53523,#53524,#53525,#53526,#53527,#53528,#53529,#53530,#53531,#53532,
#53533,#53534,#53535,#53536,#53537,#53538,#53539,#53540,#53541,#53542,#53543,
#53544,#53545,#53546,#53547,#53548,#53549,#53550,#53551,#53552,#53553,#53554,
#53555,#53556,#53557,#53558,#53559,#53560,#53561,#53562,#53563,#53564),
 .UNSPECIFIED.,.F.,.F.,(4,3,3,3,3,3,3,3,3,3,3,3,3,3,3,3,3,3,3,3,3,3,3,4),
(141.371669411541,141.468831254161,141.566438903267,141.66339620349,141.760311911022,
141.857216996242,141.955335858934,142.052368429038,142.151030438025,142.249692447012,
142.348290572016,142.446748354792,142.546970922565,142.645250480293,142.743497059367,
142.841740142405,142.943437331047,143.041821744466,143.14517532072,143.248528896974,
143.347104955699,143.445558136373,143.543900701708,143.597933925136),
 .UNSPECIFIED.);
#522=B_SPLINE_CURVE_WITH_KNOTS('',3,(#53565,#53566,#53567,#53568,#53569,
#53570,#53571,#53572),.UNSPECIFIED.,.F.,.F.,(4,1,1,1,1,4),(137.314688078281,
138.254346647165,139.253183097127,140.252019547089,141.250855997051,141.371669411541),
 .UNSPECIFIED.);
#523=B_SPLINE_CURVE_WITH_KNOTS('',3,(#53578,#53579,#53580,#53581,#53582,
#53583,#53584,#53585,#53586,#53587,#53588,#53589,#53590,#53591,#53592,#53593,
#53594,#53595,#53596,#53597,#53598,#53599,#53600,#53601,#53602,#53603,#53604,
#53605,#53606,#53607,#53608,#53609,#53610,#53611,#53612,#53613,#53614,#53615,
#53616,#53617,#53618,#53619,#53620,#53621,#53622,#53623,#53624,#53625,#53626,
#53627,#53628,#53629,#53630,#53631,#53632,#53633,#53634,#53635,#53636,#53637,
#53638,#53639,#53640,#53641,#53642,#53643,#53644,#53645,#53646,#53647,#53648,
#53649,#53650,#53651,#53652,#53653,#53654,#53655,#53656,#53657,#53658,#53659,
#53660,#53661,#53662,#53663,#53664,#53665,#53666,#53667,#53668,#53669,#53670,
#53671,#53672,#53673,#53674,#53675,#53676,#53677,#53678,#53679,#53680,#53681,
#53682,#53683,#53684,#53685,#53686,#53687,#53688,#53689,#53690,#53691,#53692,
#53693,#53694,#53695,#53696,#53697,#53698,#53699,#53700,#53701),
 .UNSPECIFIED.,.F.,.F.,(4,3,3,3,3,3,3,3,3,3,3,3,3,3,3,3,3,3,3,3,3,3,3,3,
3,3,3,3,3,3,3,3,3,3,3,3,3,3,3,3,3,4),(131.031654975012,131.129931714323,
131.228177249718,131.326421062313,131.426640354222,131.525027386608,131.62616280828,
131.727298229951,131.825896354955,131.924354137731,132.024576705504,132.122856263232,
132.221102842306,132.319345925344,132.421043113987,132.519427527405,132.622781103659,
132.726134679913,132.824732804917,132.923190587693,133.023413155466,133.121692713194,
133.219939292268,133.318182375306,133.419879563948,133.518263977367,133.621617553621,
133.724971129875,133.823569254879,133.922027037656,134.022249605428,134.120529163156,
134.21877574223,134.317018825268,134.41871601391,134.517100427329,134.620454003583,
134.723807579837,134.8363385207,134.948409000641,135.059693750753,135.088484104126),
 .UNSPECIFIED.);
#524=B_SPLINE_CURVE_WITH_KNOTS('',3,(#53702,#53703,#53704,#53705,#53706,
#53707,#53708,#53709,#53710,#53711,#53712,#53713,#53714,#53715,#53716,#53717,
#53718,#53719,#53720,#53721,#53722,#53723,#53724,#53725,#53726,#53727,#53728,
#53729,#53730,#53731,#53732,#53733,#53734,#53735,#53736,#53737,#53738,#53739,
#53740,#53741,#53742,#53743,#53744,#53745,#53746,#53747,#53748,#53749,#53750,
#53751,#53752,#53753,#53754,#53755,#53756,#53757,#53758,#53759,#53760,#53761,
#53762,#53763,#53764,#53765,#53766,#53767,#53768,#53769,#53770,#53771),
 .UNSPECIFIED.,.F.,.F.,(4,3,3,3,3,3,3,3,3,3,3,3,3,3,3,3,3,3,3,3,3,3,3,4),
(135.088484104361,135.187254556185,135.286029876603,135.384838499173,135.483776463585,
135.582788468008,135.681976179006,135.722644029799,135.821242154803,135.919699937579,
136.019922505352,136.11820206308,136.216448642154,136.314691725192,136.416388913835,
136.514773327253,136.618126903507,136.721480479761,136.820067256329,136.918521077985,
137.017401832662,137.115677672543,137.214860884617,137.314044096691),
 .UNSPECIFIED.);
#525=B_SPLINE_CURVE_WITH_KNOTS('',3,(#53773,#53774,#53775,#53776,#53777,
#53778,#53779),.UNSPECIFIED.,.F.,.F.,(4,1,1,1,4),(135.088484104361,135.257837297279,
136.256673747241,137.255510197203,137.314688078281),.UNSPECIFIED.);
#526=B_SPLINE_CURVE_WITH_KNOTS('',3,(#53780,#53781,#53782,#53783,#53784,
#53785,#53786,#53787,#53788,#53789,#53790,#53791,#53792,#53793,#53794,#53795,
#53796,#53797,#53798,#53799,#53800,#53801,#53802,#53803,#53804,#53805,#53806,
#53807,#53808,#53809,#53810,#53811,#53812,#53813,#53814,#53815,#53816,#53817,
#53818,#53819,#53820,#53821,#53822,#53823,#53824,#53825,#53826,#53827,#53828,
#53829,#53830,#53831,#53832,#53833,#53834,#53835,#53836,#53837,#53838,#53839,
#53840,#53841,#53842,#53843,#53844,#53845,#53846,#53847,#53848,#53849,#53850,
#53851,#53852,#53853,#53854,#53855,#53856,#53857,#53858,#53859,#53860,#53861,
#53862,#53863,#53864,#53865,#53866,#53867,#53868,#53869,#53870,#53871,#53872,
#53873,#53874,#53875,#53876,#53877,#53878,#53879,#53880,#53881,#53882,#53883,
#53884,#53885,#53886,#53887,#53888,#53889,#53890,#53891,#53892,#53893,#53894,
#53895,#53896,#53897,#53898,#53899,#53900,#53901,#53902,#53903,#53904,#53905,
#53906),.UNSPECIFIED.,.F.,.F.,(4,3,3,3,3,3,3,3,3,3,3,3,3,3,3,3,3,3,3,3,
3,3,3,3,3,3,3,3,3,3,3,3,3,3,3,3,3,3,3,3,3,3,4),(131.030544946366,131.128979442315,
131.227573135221,131.262491497432,131.361089622436,131.459547405213,131.559769972985,
131.658049530713,131.756296109787,131.854539192825,131.956236381468,132.054620794886,
132.15797437114,132.261327947394,132.359926072398,132.458383855174,132.558606422947,
132.656885980675,132.755132559749,132.853375642787,132.955072831429,133.053457244848,
133.156810821102,133.260164397356,133.35876252236,133.457220305136,133.557442872909,
133.655722430637,133.75396900971,133.852212092749,133.953909281391,134.05229369481,
134.155647271063,134.259000847317,134.356128675186,134.453094160804,134.549968416922,
134.646782617699,134.743567858737,134.840399971759,134.937256811785,135.034231214224,
135.088484104361),.UNSPECIFIED.);
#527=B_SPLINE_CURVE_WITH_KNOTS('',3,(#53912,#53913,#53914,#53915,#53916,
#53917,#53918,#53919),.UNSPECIFIED.,.F.,.F.,(4,1,1,1,1,4),(124.74803348566,
125.73427953018,126.733115980142,127.731952430104,128.730788880066,128.805298797182),
 .UNSPECIFIED.);
#528=B_SPLINE_CURVE_WITH_KNOTS('',3,(#53920,#53921,#53922,#53923,#53924,
#53925,#53926,#53927,#53928,#53929,#53930,#53931,#53932,#53933,#53934,#53935,
#53936,#53937,#53938,#53939,#53940,#53941,#53942,#53943,#53944,#53945,#53946,
#53947,#53948,#53949,#53950,#53951,#53952,#53953,#53954,#53955,#53956,#53957,
#53958,#53959,#53960,#53961,#53962,#53963,#53964,#53965,#53966,#53967,#53968,
#53969,#53970,#53971,#53972,#53973,#53974,#53975,#53976,#53977,#53978,#53979,
#53980,#53981,#53982,#53983,#53984,#53985,#53986,#53987,#53988,#53989),
 .UNSPECIFIED.,.F.,.F.,(4,3,3,3,3,3,3,3,3,3,3,3,3,3,3,3,3,3,3,3,3,3,3,4),
(128.805298797182,128.902840431273,129.000250613517,129.097560812666,129.194818343698,
129.292053887497,129.389298094495,129.486642967568,129.584044330746,129.68160592498,
129.729625330028,129.828223455032,129.926681237808,130.026903805581,130.125183363309,
130.223429942382,130.321673025421,130.423370214063,130.521754627482,130.625108203735,
130.728461779989,130.82704702784,130.929351001426,131.031654975012),
 .UNSPECIFIED.);
#529=B_SPLINE_CURVE_WITH_KNOTS('',3,(#53991,#53992,#53993,#53994,#53995,
#53996,#53997,#53998,#53999,#54000,#54001,#54002,#54003,#54004,#54005,#54006,
#54007,#54008,#54009,#54010,#54011,#54012,#54013,#54014,#54015,#54016,#54017,
#54018,#54019,#54020,#54021,#54022,#54023,#54024,#54025,#54026,#54027,#54028,
#54029,#54030,#54031,#54032,#54033,#54034,#54035,#54036,#54037,#54038,#54039,
#54040,#54041,#54042,#54043,#54044,#54045,#54046,#54047,#54048,#54049,#54050,
#54051,#54052,#54053,#54054,#54055,#54056,#54057,#54058,#54059,#54060),
 .UNSPECIFIED.,.F.,.F.,(4,3,3,3,3,3,3,3,3,3,3,3,3,3,3,3,3,3,3,3,3,3,3,4),
(128.80529901116,128.910085619871,129.015255759151,129.120630109632,129.226318351047,
129.264818597508,129.363416722512,129.461874505288,129.562097073061,129.660376630789,
129.758623209863,129.856866292901,129.958563481543,130.056947894962,130.160301471216,
130.26365504747,130.362225486655,130.460667523599,130.55901086589,130.657285118175,
130.755545076206,130.853792579363,130.952108672699,131.030544946366),
 .UNSPECIFIED.);
#530=B_SPLINE_CURVE_WITH_KNOTS('',3,(#54061,#54062,#54063,#54064,#54065,
#54066,#54067,#54068),.UNSPECIFIED.,.F.,.F.,(4,1,1,1,1,4),(124.748072442403,
125.269472797661,126.268309247622,127.267145697584,128.265982147546,128.805298797182),
 .UNSPECIFIED.);
#531=B_SPLINE_CURVE_WITH_KNOTS('',3,(#54074,#54075,#54076,#54077,#54078,
#54079,#54080,#54081,#54082,#54083,#54084,#54085,#54086,#54087,#54088,#54089,
#54090,#54091,#54092,#54093,#54094,#54095,#54096,#54097,#54098,#54099,#54100,
#54101,#54102,#54103,#54104,#54105,#54106,#54107,#54108,#54109,#54110,#54111,
#54112,#54113,#54114,#54115,#54116,#54117,#54118,#54119,#54120,#54121,#54122,
#54123,#54124,#54125,#54126,#54127,#54128,#54129,#54130,#54131,#54132,#54133,
#54134,#54135,#54136,#54137,#54138,#54139,#54140,#54141,#54142,#54143,#54144,
#54145,#54146,#54147,#54148,#54149,#54150,#54151,#54152,#54153,#54154,#54155,
#54156,#54157,#54158,#54159,#54160,#54161,#54162,#54163,#54164,#54165,#54166,
#54167,#54168,#54169,#54170,#54171,#54172,#54173,#54174,#54175,#54176,#54177,
#54178,#54179,#54180,#54181,#54182,#54183,#54184,#54185,#54186,#54187,#54188,
#54189,#54190,#54191,#54192,#54193,#54194,#54195,#54196,#54197),
 .UNSPECIFIED.,.F.,.F.,(4,3,3,3,3,3,3,3,3,3,3,3,3,3,3,3,3,3,3,3,3,3,3,3,
3,3,3,3,3,3,3,3,3,3,3,3,3,3,3,3,3,4),(118.464214610255,118.562615728343,
118.661189998764,118.742424380447,118.841022505451,118.939480288228,119.039702856,
119.137982413728,119.236228992802,119.33447207584,119.436169264482,119.534553677901,
119.637907254155,119.741260830409,119.839858955413,119.93831673819,120.038539305963,
120.136818863691,120.235065442764,120.333308525802,120.435005714445,120.533390127863,
120.636743704117,120.740097280371,120.838695405375,120.937153188151,121.037375755924,
121.135655313652,121.233901892726,121.332144975764,121.433842164407,121.532226577825,
121.635580154079,121.738933730333,121.836831200292,121.933909156543,122.030894120917,
122.127817176647,122.226391254986,122.323316910845,122.422715200424,122.522113490002),
 .UNSPECIFIED.);
#532=B_SPLINE_CURVE_WITH_KNOTS('',3,(#54198,#54199,#54200,#54201,#54202,
#54203,#54204),.UNSPECIFIED.,.F.,.F.,(4,1,1,1,4),(122.522113490002,122.737770180294,
123.736606630256,124.735443080218,124.74803348566),.UNSPECIFIED.);
#533=B_SPLINE_CURVE_WITH_KNOTS('',3,(#54206,#54207,#54208,#54209,#54210,
#54211),.UNSPECIFIED.,.F.,.F.,(4,1,1,4),(122.522113490002,123.271799897737,
124.270636347699,124.748072442403),.UNSPECIFIED.);
#534=B_SPLINE_CURVE_WITH_KNOTS('',3,(#54212,#54213,#54214,#54215,#54216,
#54217,#54218,#54219,#54220,#54221,#54222,#54223,#54224,#54225,#54226,#54227,
#54228,#54229,#54230,#54231,#54232,#54233,#54234,#54235,#54236,#54237,#54238,
#54239,#54240,#54241,#54242,#54243,#54244,#54245,#54246,#54247,#54248,#54249,
#54250,#54251,#54252,#54253,#54254,#54255,#54256,#54257,#54258,#54259,#54260,
#54261,#54262,#54263,#54264,#54265,#54266,#54267,#54268,#54269,#54270,#54271,
#54272,#54273,#54274,#54275,#54276,#54277,#54278,#54279,#54280,#54281,#54282,
#54283,#54284,#54285,#54286,#54287,#54288,#54289,#54290,#54291,#54292,#54293,
#54294,#54295,#54296,#54297,#54298,#54299,#54300,#54301,#54302,#54303,#54304,
#54305,#54306,#54307,#54308,#54309,#54310,#54311,#54312,#54313,#54314,#54315,
#54316,#54317,#54318,#54319,#54320,#54321,#54322,#54323,#54324,#54325,#54326,
#54327,#54328,#54329,#54330,#54331,#54332,#54333,#54334,#54335),
 .UNSPECIFIED.,.F.,.F.,(4,3,3,3,3,3,3,3,3,3,3,3,3,3,3,3,3,3,3,3,3,3,3,3,
3,3,3,3,3,3,3,3,3,3,3,3,3,3,3,3,3,4),(118.465360151754,118.566746895021,
118.66503051079,118.763278702571,118.861520955212,118.959786738854,119.05816456808,
119.156610036517,119.255210841691,119.276454097889,119.375052222893,119.47351000567,
119.573732573442,119.67201213117,119.770258710244,119.868501793282,119.970198981925,
120.068583395343,120.171936971597,120.275290547851,120.373888672855,120.472346455631,
120.572569023404,120.670848581132,120.769095160206,120.867338243244,120.969035431886,
121.067419845305,121.170773421559,121.274126997813,121.372725122817,121.471182905593,
121.571405473366,121.669685031094,121.767931610168,121.866174693206,121.967871881848,
122.066256295267,122.169609871521,122.272963447775,122.400857829821,122.52211338997),
 .UNSPECIFIED.);
#535=B_SPLINE_CURVE_WITH_KNOTS('',3,(#54341,#54342,#54343,#54344,#54345,
#54346,#54347,#54348,#54349,#54350,#54351,#54352,#54353,#54354,#54355,#54356,
#54357,#54358,#54359,#54360,#54361,#54362,#54363,#54364,#54365,#54366,#54367,
#54368,#54369,#54370,#54371,#54372,#54373,#54374,#54375,#54376,#54377,#54378,
#54379,#54380,#54381,#54382,#54383,#54384,#54385,#54386,#54387,#54388,#54389,
#54390,#54391,#54392,#54393,#54394,#54395,#54396,#54397,#54398,#54399,#54400,
#54401,#54402,#54403,#54404,#54405,#54406,#54407,#54408,#54409,#54410,#54411,
#54412,#54413,#54414,#54415,#54416,#54417,#54418,#54419,#54420,#54421,#54422,
#54423,#54424,#54425,#54426,#54427,#54428,#54429,#54430,#54431,#54432,#54433,
#54434,#54435,#54436,#54437,#54438,#54439,#54440,#54441,#54442,#54443,#54444,
#54445,#54446,#54447,#54448,#54449,#54450,#54451,#54452,#54453,#54454,#54455,
#54456,#54457,#54458,#54459,#54460,#54461,#54462,#54463,#54464),
 .UNSPECIFIED.,.F.,.F.,(4,3,3,3,3,3,3,3,3,3,3,3,3,3,3,3,3,3,3,3,3,3,3,3,
3,3,3,3,3,3,3,3,3,3,3,3,3,3,3,3,3,4),(112.181790934622,112.280032837375,
112.378281941166,112.476633717368,112.575038455028,112.673614634251,112.749405680676,
112.84800380568,112.946461588457,113.046684156229,113.144963713957,113.243210293031,
113.341453376069,113.443150564711,113.54153497813,113.644888554384,113.748242130638,
113.846840255642,113.945298038418,114.045520606191,114.143800163919,114.242046742992,
114.34028982603,114.441987014673,114.540371428091,114.643725004345,114.747078580599,
114.845676705603,114.944134488379,115.044357056152,115.14263661388,115.240883192953,
115.339126275992,115.440823464634,115.539207878053,115.642561454307,115.745915030561,
115.849888759331,115.953561696348,116.057054365164,116.160309146371,116.238928182547),
 .UNSPECIFIED.);
#536=B_SPLINE_CURVE_WITH_KNOTS('',3,(#54465,#54466,#54467,#54468,#54469,
#54470,#54471,#54472,#54473,#54474,#54475,#54476,#54477,#54478,#54479,#54480,
#54481,#54482,#54483,#54484,#54485,#54486,#54487,#54488,#54489,#54490,#54491,
#54492,#54493,#54494,#54495,#54496,#54497,#54498,#54499,#54500,#54501,#54502,
#54503,#54504,#54505,#54506,#54507,#54508,#54509,#54510,#54511,#54512,#54513,
#54514,#54515,#54516,#54517,#54518,#54519,#54520,#54521,#54522,#54523,#54524,
#54525,#54526,#54527,#54528,#54529,#54530,#54531,#54532,#54533,#54534),
 .UNSPECIFIED.,.F.,.F.,(4,3,3,3,3,3,3,3,3,3,3,3,3,3,3,3,3,3,3,3,3,3,3,4),
(116.238928182823,116.341566510357,116.44447107289,116.547509821617,116.650828963887,
116.744751480523,116.843349605527,116.941807388303,117.042029956076,117.140309513804,
117.238556092877,117.336799175916,117.438496364558,117.536880777977,117.640234354231,
117.743587930485,117.842162082216,117.940606624237,118.038951269659,118.137225626952,
118.235476585644,118.333714612383,118.431998836548,118.464214610255),
 .UNSPECIFIED.);
#537=B_SPLINE_CURVE_WITH_KNOTS('',3,(#54536,#54537,#54538,#54539,#54540,
#54541,#54542,#54543,#54544,#54545,#54546,#54547,#54548,#54549,#54550,#54551,
#54552,#54553,#54554,#54555,#54556,#54557,#54558,#54559,#54560,#54561,#54562,
#54563,#54564,#54565,#54566,#54567,#54568,#54569,#54570,#54571,#54572,#54573,
#54574,#54575,#54576,#54577,#54578,#54579,#54580,#54581,#54582,#54583,#54584,
#54585,#54586,#54587,#54588,#54589,#54590,#54591,#54592,#54593,#54594,#54595,
#54596,#54597,#54598,#54599,#54600,#54601,#54602,#54603,#54604,#54605),
 .UNSPECIFIED.,.F.,.F.,(4,3,3,3,3,3,3,3,3,3,3,3,3,3,3,3,3,3,3,3,3,3,3,4),
(116.238928182823,116.279944748004,116.378542873008,116.477000655784,116.577223223557,
116.675502781285,116.773749360358,116.871992443397,116.973689632039,117.072074045458,
117.175427621712,117.278781197966,117.37737932297,117.475837105746,117.576059673519,
117.674339231247,117.77258581032,117.870828893359,117.972526082001,118.07091049542,
118.174264071673,118.277617647927,118.376189313834,118.465360151754),
 .UNSPECIFIED.);
#538=B_SPLINE_CURVE_WITH_KNOTS('',3,(#54606,#54607,#54608,#54609,#54610,
#54611,#54612,#54613),.UNSPECIFIED.,.F.,.F.,(4,1,1,1,1,4),(112.180986330182,
112.284598948156,113.283435398118,114.28227184808,115.281108298042,116.238922797526),
 .UNSPECIFIED.);
#539=B_SPLINE_CURVE_WITH_KNOTS('',3,(#54619,#54620,#54621,#54622,#54623,
#54624,#54625,#54626,#54627,#54628,#54629,#54630,#54631,#54632,#54633,#54634,
#54635,#54636,#54637,#54638,#54639,#54640,#54641,#54642,#54643,#54644,#54645,
#54646,#54647,#54648,#54649,#54650,#54651,#54652,#54653,#54654,#54655,#54656,
#54657,#54658,#54659,#54660,#54661,#54662,#54663,#54664,#54665,#54666,#54667,
#54668,#54669,#54670,#54671,#54672,#54673,#54674,#54675,#54676,#54677,#54678,
#54679,#54680,#54681,#54682,#54683,#54684,#54685,#54686,#54687,#54688,#54689,
#54690,#54691,#54692,#54693,#54694,#54695,#54696,#54697,#54698,#54699,#54700,
#54701,#54702,#54703,#54704,#54705,#54706,#54707,#54708,#54709,#54710,#54711,
#54712,#54713,#54714,#54715,#54716,#54717,#54718,#54719,#54720,#54721,#54722,
#54723,#54724,#54725,#54726,#54727,#54728,#54729,#54730,#54731,#54732,#54733,
#54734,#54735,#54736,#54737,#54738,#54739,#54740,#54741,#54742),
 .UNSPECIFIED.,.F.,.F.,(4,3,3,3,3,3,3,3,3,3,3,3,3,3,3,3,3,3,3,3,3,3,3,3,
3,3,3,3,3,3,3,3,3,3,3,3,3,3,3,3,3,4),(105.898938930965,105.997345977956,
106.095658486362,106.193920763664,106.292162312088,106.390412605836,106.488766498079,
106.587174739352,106.685752818818,106.756386980905,106.854985105909,106.953442888685,
107.053665456458,107.151945014186,107.250191593259,107.348434676298,107.45013186494,
107.548516278359,107.651869854612,107.755223430866,107.85382155587,107.952279338646,
108.052501906419,108.150781464147,108.24902804322,108.347271126259,108.448968314901,
108.54735272832,108.650706304574,108.754059880828,108.852658005832,108.951115788608,
109.051338356381,109.149617914109,109.247864493183,109.346107576221,109.447804764863,
109.546189178282,109.649542754536,109.75289633079,109.893212936346,109.955742875643),
 .UNSPECIFIED.);
#540=B_SPLINE_CURVE_WITH_KNOTS('',3,(#54743,#54744,#54745,#54746,#54747,
#54748,#54749,#54750,#54751,#54752,#54753,#54754,#54755,#54756,#54757,#54758,
#54759,#54760,#54761,#54762,#54763,#54764,#54765,#54766,#54767,#54768,#54769,
#54770,#54771,#54772,#54773,#54774,#54775,#54776,#54777,#54778,#54779,#54780,
#54781,#54782,#54783,#54784,#54785,#54786,#54787,#54788,#54789,#54790,#54791,
#54792,#54793,#54794,#54795,#54796,#54797,#54798,#54799,#54800,#54801,#54802,
#54803,#54804,#54805,#54806,#54807,#54808,#54809,#54810,#54811,#54812,#54813,
#54814,#54815),.UNSPECIFIED.,.F.,.F.,(4,3,3,3,3,3,3,3,3,3,3,3,3,3,3,3,3,
3,3,3,3,3,3,3,4),(109.955742875951,110.055241614051,110.152151423466,110.249014842069,
110.345862894414,110.447330365999,110.544300028994,110.641334438529,110.738518045248,
110.751732780752,110.850330905756,110.948788688533,111.049011256305,111.147290814034,
111.245537393107,111.343780476145,111.445477664788,111.543862078206,111.64721565446,
111.750569230714,111.849176820414,111.947618966285,112.045965736407,112.144240689691,
112.181790934622),.UNSPECIFIED.);
#541=B_SPLINE_CURVE_WITH_KNOTS('',3,(#54817,#54818,#54819,#54820,#54821,
#54822),.UNSPECIFIED.,.F.,.F.,(4,1,1,4),(109.955750010146,110.286926048232,
111.285762498194,112.180986330182),.UNSPECIFIED.);
#542=B_SPLINE_CURVE_WITH_KNOTS('',3,(#54823,#54824,#54825,#54826,#54827,
#54828,#54829,#54830,#54831,#54832,#54833,#54834,#54835,#54836,#54837,#54838,
#54839,#54840,#54841,#54842,#54843,#54844,#54845,#54846,#54847,#54848,#54849,
#54850,#54851,#54852,#54853,#54854,#54855,#54856,#54857,#54858,#54859,#54860,
#54861,#54862,#54863,#54864,#54865,#54866,#54867,#54868,#54869,#54870,#54871,
#54872,#54873,#54874,#54875,#54876,#54877,#54878,#54879,#54880,#54881,#54882,
#54883,#54884,#54885,#54886,#54887,#54888,#54889,#54890,#54891,#54892,#54893,
#54894,#54895,#54896,#54897,#54898,#54899,#54900,#54901,#54902,#54903,#54904,
#54905,#54906,#54907,#54908,#54909,#54910,#54911,#54912,#54913,#54914,#54915,
#54916,#54917,#54918,#54919,#54920,#54921,#54922,#54923,#54924,#54925,#54926,
#54927,#54928,#54929,#54930,#54931,#54932,#54933,#54934,#54935,#54936,#54937,
#54938,#54939,#54940,#54941,#54942,#54943,#54944,#54945,#54946),
 .UNSPECIFIED.,.F.,.F.,(4,3,3,3,3,3,3,3,3,3,3,3,3,3,3,3,3,3,3,3,3,3,3,3,
3,3,3,3,3,3,3,3,3,3,3,3,3,3,3,3,3,4),(105.898082547599,105.996456972795,
106.094847349944,106.193416320635,106.291580248385,106.390178373389,106.488636156166,
106.588858723938,106.687138281666,106.78538486074,106.883627943778,106.985325132421,
107.083709545839,107.187063122093,107.290416698347,107.389014823351,107.487472606128,
107.5876951739,107.685974731629,107.784221310702,107.88246439374,107.984161582382,
108.082545995801,108.185899572055,108.289253148309,108.387851273313,108.486309056089,
108.586531623862,108.68481118159,108.783057760664,108.881300843702,108.982998032344,
109.081382445763,109.184736022017,109.288089598271,109.386591328535,109.484956309732,
109.583214317041,109.681399820023,109.779540599733,109.877698313764,109.955742875643),
 .UNSPECIFIED.);
#543=B_SPLINE_CURVE_WITH_KNOTS('',3,(#54952,#54953,#54954,#54955,#54956,
#54957,#54958,#54959),.UNSPECIFIED.,.F.,.F.,(4,1,1,1,1,4),(99.6144332356559,
99.7645318311714,100.763368281133,101.762204731095,102.761041181057,103.672548858943),
 .UNSPECIFIED.);
#544=B_SPLINE_CURVE_WITH_KNOTS('',3,(#54960,#54961,#54962,#54963,#54964,
#54965,#54966,#54967,#54968,#54969,#54970,#54971,#54972,#54973,#54974,#54975,
#54976,#54977,#54978,#54979,#54980,#54981,#54982,#54983,#54984,#54985,#54986,
#54987,#54988,#54989,#54990,#54991,#54992,#54993,#54994,#54995,#54996,#54997,
#54998,#54999,#55000,#55001,#55002,#55003,#55004,#55005,#55006,#55007,#55008,
#55009,#55010,#55011,#55012,#55013,#55014,#55015,#55016,#55017,#55018,#55019,
#55020,#55021,#55022,#55023,#55024,#55025,#55026,#55027,#55028,#55029),
 .UNSPECIFIED.,.F.,.F.,(4,3,3,3,3,3,3,3,3,3,3,3,3,3,3,3,3,3,3,3,3,3,3,4),
(103.672557568463,103.759877631019,103.858475756023,103.9569335388,104.057156106572,
104.1554356643,104.253682243374,104.351925326412,104.453622515054,104.552006928473,
104.655360504727,104.758714080981,104.857312205985,104.955769988762,105.055992556534,
105.154272114262,105.252518693336,105.350761776374,105.452458965017,105.550843378435,
105.654196954689,105.757550530943,105.856140410583,105.898938930965),
 .UNSPECIFIED.);
#545=B_SPLINE_CURVE_WITH_KNOTS('',3,(#55031,#55032,#55033,#55034,#55035,
#55036,#55037,#55038,#55039,#55040,#55041,#55042,#55043,#55044,#55045,#55046,
#55047,#55048,#55049,#55050,#55051,#55052,#55053,#55054,#55055,#55056,#55057,
#55058,#55059,#55060,#55061,#55062,#55063,#55064,#55065,#55066,#55067,#55068,
#55069,#55070,#55071,#55072,#55073,#55074,#55075,#55076,#55077,#55078,#55079,
#55080,#55081,#55082,#55083,#55084,#55085,#55086,#55087,#55088,#55089,#55090,
#55091,#55092,#55093,#55094,#55095,#55096,#55097,#55098,#55099,#55100,#55101,
#55102,#55103),.UNSPECIFIED.,.F.,.F.,(4,3,3,3,3,3,3,3,3,3,3,3,3,3,3,3,3,
3,3,3,3,3,3,3,4),(103.672557568463,103.771601702603,103.870660322484,103.96976131202,
104.06899945985,104.168318657834,104.267812431338,104.293907348461,104.392505473465,
104.490963256241,104.591185824014,104.689465381742,104.787711960816,104.885955043854,
104.987652232496,105.086036645915,105.189390222169,105.292743798423,105.39132916073,
105.489781902009,105.591857063406,105.690131970176,105.788367325635,105.886604359972,
105.898082547599),.UNSPECIFIED.);
#546=B_SPLINE_CURVE_WITH_KNOTS('',3,(#55104,#55105,#55106,#55107,#55108,
#55109,#55110,#55111),.UNSPECIFIED.,.F.,.F.,(4,1,1,1,1,4),(99.616027896677,
100.298561548614,101.297397998576,102.296234448537,103.295070898499,103.672550060648),
 .UNSPECIFIED.);
#547=B_SPLINE_CURVE_WITH_KNOTS('',3,(#55117,#55118,#55119,#55120,#55121,
#55122,#55123,#55124,#55125,#55126,#55127,#55128,#55129,#55130,#55131,#55132,
#55133,#55134,#55135,#55136,#55137,#55138,#55139,#55140,#55141,#55142,#55143,
#55144,#55145,#55146,#55147,#55148,#55149,#55150,#55151,#55152,#55153,#55154,
#55155,#55156,#55157,#55158,#55159,#55160,#55161,#55162,#55163,#55164,#55165,
#55166,#55167,#55168,#55169,#55170,#55171,#55172,#55173,#55174,#55175,#55176,
#55177,#55178,#55179,#55180,#55181,#55182,#55183,#55184,#55185,#55186,#55187,
#55188,#55189,#55190,#55191,#55192,#55193,#55194,#55195,#55196,#55197,#55198,
#55199,#55200,#55201,#55202,#55203,#55204,#55205,#55206,#55207,#55208,#55209,
#55210,#55211,#55212,#55213,#55214,#55215,#55216,#55217,#55218,#55219,#55220,
#55221,#55222,#55223,#55224,#55225,#55226,#55227,#55228,#55229,#55230,#55231,
#55232,#55233,#55234,#55235,#55236,#55237,#55238,#55239,#55240,#55241,#55242,
#55243),.UNSPECIFIED.,.F.,.F.,(4,3,3,3,3,3,3,3,3,3,3,3,3,3,3,3,3,3,3,3,
3,3,3,3,3,3,3,3,3,3,3,3,3,3,3,3,3,3,3,3,3,3,4),(93.3318434577557,93.430100540662,
93.5284655250177,93.6268914778956,93.7254798525794,93.7715131314001,93.8701112564038,
93.9685690391807,94.0687916069534,94.1670711646815,94.2653177437549,94.3635608267937,
94.4652580154358,94.5636424288546,94.6669960051083,94.770349581362,94.8689477063657,
94.9674054891427,95.0676280569154,95.1659076146435,95.264154193717,95.3623972767553,
95.4640944653975,95.5624788788163,95.6658324550701,95.7691860313239,95.8677841563275,
95.9662419391041,96.0664645068768,96.164744064605,96.2629906436783,96.361233726717,
96.4629309153592,96.5613153287781,96.6646689050319,96.7680224812858,96.8674993725788,
96.9668292609825,97.0660403563896,97.1651524247991,97.2642075332237,97.3632407686266,
97.3893722612837),.UNSPECIFIED.);
#548=B_SPLINE_CURVE_WITH_KNOTS('',3,(#55244,#55245,#55246,#55247,#55248,
#55249),.UNSPECIFIED.,.F.,.F.,(4,1,1,4),(97.3893797695142,97.7668589312476,
98.7656953812095,99.6144332356559),.UNSPECIFIED.);
#549=B_SPLINE_CURVE_WITH_KNOTS('',3,(#55251,#55252,#55253,#55254,#55255,
#55256),.UNSPECIFIED.,.F.,.F.,(4,1,1,4),(97.3893809712563,98.3008886486899,
99.2997250986518,99.616027896677),.UNSPECIFIED.);
#550=B_SPLINE_CURVE_WITH_KNOTS('',3,(#55257,#55258,#55259,#55260,#55261,
#55262,#55263,#55264,#55265,#55266,#55267,#55268,#55269,#55270,#55271,#55272,
#55273,#55274,#55275,#55276,#55277,#55278,#55279,#55280,#55281,#55282,#55283,
#55284,#55285,#55286,#55287,#55288,#55289,#55290,#55291,#55292,#55293,#55294,
#55295,#55296,#55297,#55298,#55299,#55300,#55301,#55302,#55303,#55304,#55305,
#55306,#55307,#55308,#55309,#55310,#55311,#55312,#55313,#55314,#55315,#55316,
#55317,#55318,#55319,#55320,#55321,#55322,#55323,#55324,#55325,#55326,#55327,
#55328,#55329,#55330,#55331,#55332,#55333,#55334,#55335,#55336,#55337,#55338,
#55339,#55340,#55341,#55342,#55343,#55344,#55345,#55346,#55347,#55348,#55349,
#55350,#55351,#55352,#55353,#55354,#55355,#55356,#55357,#55358,#55359,#55360,
#55361,#55362,#55363,#55364,#55365,#55366,#55367,#55368,#55369,#55370,#55371,
#55372,#55373,#55374,#55375,#55376,#55377,#55378,#55379,#55380),
 .UNSPECIFIED.,.F.,.F.,(4,3,3,3,3,3,3,3,3,3,3,3,3,3,3,3,3,3,3,3,3,3,3,3,
3,3,3,3,3,3,3,3,3,3,3,3,3,3,3,3,3,4),(93.3321733295568,93.4307320757135,
93.5291589669388,93.6274833960061,93.725752386932,93.8239954496423,93.9222420613545,
94.0205891224222,94.1189858639191,94.2175579055399,94.3055428488424,94.4041409738461,
94.5025987566229,94.6028213243955,94.7011008821237,94.7993474611971,94.8975905442356,
94.9992877328778,95.0976721462966,95.2010257225504,95.3043792988043,95.402977423808,
95.5014352065848,95.6016577743575,95.6999373320856,95.798183911159,95.8964269941974,
95.9981241828396,96.0965085962584,96.1998621725123,96.3032157487662,96.4018138737699,
96.5002716565466,96.6004942243193,96.6987737820475,96.7970203611208,96.8952634441593,
96.9969606328015,97.0953450462203,97.1986986224741,97.302052198728,97.3893722612837),
 .UNSPECIFIED.);
#551=B_SPLINE_CURVE_WITH_KNOTS('',3,(#55386,#55387,#55388,#55389,#55390,
#55391,#55392,#55393),.UNSPECIFIED.,.F.,.F.,(4,1,1,1,1,4),(87.049742935369,
87.7784944316289,88.7773308815908,89.7761673315526,90.7750037815145,91.1061798190633),
 .UNSPECIFIED.);
#552=B_SPLINE_CURVE_WITH_KNOTS('',3,(#55394,#55395,#55396,#55397,#55398,
#55399,#55400,#55401,#55402,#55403,#55404,#55405,#55406,#55407,#55408,#55409,
#55410,#55411,#55412,#55413,#55414,#55415,#55416,#55417,#55418,#55419,#55420,
#55421,#55422,#55423,#55424,#55425,#55426,#55427,#55428,#55429,#55430,#55431,
#55432,#55433,#55434,#55435,#55436,#55437,#55438,#55439,#55440,#55441,#55442,
#55443,#55444,#55445,#55446,#55447,#55448,#55449,#55450,#55451,#55452,#55453,
#55454,#55455,#55456,#55457,#55458,#55459,#55460,#55461,#55462,#55463),
 .UNSPECIFIED.,.F.,.F.,(4,3,3,3,3,3,3,3,3,3,3,3,3,3,3,3,3,3,3,3,3,3,3,4),
(91.1061869541041,91.204341964477,91.3024795334307,91.4006291648839,91.4988897541856,
91.5972075103077,91.6957053368613,91.7738402314764,91.8724383564801,91.9708961392568,
92.0711187070294,92.1693982647576,92.2676448438311,92.3658879268697,92.4675851155119,
92.5659695289307,92.6693231051845,92.7726766814383,92.8712673172515,92.9697241251222,
93.0680663331333,93.1663410384397,93.2645927043656,93.3318434577557),
 .UNSPECIFIED.);
#553=B_SPLINE_CURVE_WITH_KNOTS('',3,(#55465,#55466,#55467,#55468,#55469,
#55470,#55471,#55472,#55473,#55474,#55475,#55476,#55477,#55478,#55479,#55480,
#55481,#55482,#55483,#55484,#55485,#55486,#55487,#55488,#55489,#55490,#55491,
#55492,#55493,#55494,#55495,#55496,#55497,#55498,#55499,#55500,#55501,#55502,
#55503,#55504,#55505,#55506,#55507,#55508,#55509,#55510,#55511,#55512,#55513,
#55514,#55515,#55516,#55517,#55518,#55519,#55520,#55521,#55522,#55523,#55524,
#55525,#55526,#55527,#55528,#55529,#55530,#55531,#55532,#55533,#55534),
 .UNSPECIFIED.,.F.,.F.,(4,3,3,3,3,3,3,3,3,3,3,3,3,3,3,3,3,3,3,3,3,3,3,4),
(91.1061869541041,91.246503559673,91.3090334989568,91.4076316239605,91.5060894067373,
91.6063119745099,91.7045915322381,91.8028381113116,91.9010811943501,92.0027783829923,
92.101162796411,92.2045163726649,92.3078699489187,92.4064680739224,92.5049258566991,
92.6051484244718,92.7034279822,92.8016745612733,92.8999176443118,93.001614832954,
93.0999992463728,93.2033528226267,93.3067063988806,93.3321733295568),
 .UNSPECIFIED.);
#554=B_SPLINE_CURVE_WITH_KNOTS('',3,(#55535,#55536,#55537,#55538,#55539,
#55540,#55541,#55542,#55543,#55544,#55545,#55546,#55547,#55548,#55549,#55550,
#55551,#55552,#55553,#55554,#55555,#55556,#55557,#55558,#55559,#55560,#55561,
#55562,#55563,#55564,#55565,#55566,#55567,#55568,#55569,#55570,#55571,#55572,
#55573,#55574,#55575,#55576,#55577,#55578,#55579,#55580,#55581,#55582,#55583,
#55584,#55585,#55586,#55587,#55588,#55589,#55590,#55591,#55592,#55593,#55594,
#55595,#55596,#55597,#55598,#55599,#55600,#55601,#55602,#55603,#55604,#55605,
#55606,#55607,#55608,#55609,#55610,#55611,#55612,#55613,#55614,#55615,#55616,
#55617,#55618,#55619,#55620,#55621,#55622,#55623,#55624,#55625,#55626,#55627,
#55628,#55629,#55630,#55631,#55632,#55633,#55634,#55635,#55636,#55637,#55638,
#55639,#55640,#55641,#55642,#55643,#55644,#55645,#55646,#55647,#55648,#55649,
#55650,#55651,#55652,#55653,#55654,#55655,#55656,#55657,#55658,#55659,#55660,
#55661),.UNSPECIFIED.,.F.,.F.,(4,3,3,3,3,3,3,3,3,3,3,3,3,3,3,3,3,3,3,3,
3,3,3,3,3,3,3,3,3,3,3,3,3,3,3,3,3,3,3,3,3,3,4),(87.0482730730921,87.1466828368096,
87.2452617573112,87.3136876991093,87.412285824113,87.5107436068897,87.6109661746624,
87.7092457323906,87.807492311464,87.9057353945025,88.0074325831447,88.1058169965635,
88.2091705728173,88.3125241490712,88.4111222740749,88.5095800568516,88.6098026246243,
88.7080821823524,88.8063287614258,88.9045718444643,89.0062690331065,89.1046534465253,
89.2080070227792,89.3113605990331,89.4099587240368,89.5084165068135,89.6086390745862,
89.7069186323143,89.8051652113877,89.9034082944262,90.0051054830684,90.1034898964872,
90.206843472741,90.3101970489949,90.409695787095,90.5067185530535,90.6036495481491,
90.7005198981799,90.801936662084,90.8988156754797,90.9957205549586,91.0927209416412,
91.1061869537961),.UNSPECIFIED.);
#555=B_SPLINE_CURVE_WITH_KNOTS('',3,(#55667,#55668,#55669,#55670,#55671,
#55672,#55673,#55674,#55675,#55676,#55677,#55678,#55679,#55680,#55681,#55682,
#55683,#55684,#55685,#55686,#55687,#55688,#55689,#55690,#55691,#55692,#55693,
#55694,#55695,#55696,#55697,#55698,#55699,#55700,#55701,#55702,#55703,#55704,
#55705,#55706,#55707,#55708,#55709,#55710,#55711,#55712,#55713,#55714,#55715,
#55716,#55717,#55718,#55719,#55720,#55721,#55722,#55723,#55724,#55725,#55726,
#55727,#55728,#55729,#55730,#55731,#55732,#55733,#55734,#55735,#55736,#55737,
#55738,#55739,#55740,#55741,#55742,#55743,#55744,#55745,#55746,#55747,#55748,
#55749,#55750,#55751,#55752,#55753,#55754,#55755,#55756,#55757,#55758,#55759,
#55760,#55761,#55762,#55763,#55764,#55765,#55766,#55767,#55768,#55769,#55770,
#55771,#55772,#55773,#55774,#55775,#55776,#55777,#55778,#55779,#55780,#55781,
#55782,#55783,#55784,#55785,#55786,#55787,#55788,#55789,#55790,#55791,#55792,
#55793),.UNSPECIFIED.,.F.,.F.,(4,3,3,3,3,3,3,3,3,3,3,3,3,3,3,3,3,3,3,3,
3,3,3,3,3,3,3,3,3,3,3,3,3,3,3,3,3,3,3,3,3,3,4),(80.7655329655535,80.7866392818958,
80.8852374068995,80.9836951896763,81.0839177574489,81.1821973151771,81.2804438942505,
81.378686977289,81.4803841659311,81.57876857935,81.6821221556038,81.7854757318576,
81.8840738568613,81.982531639638,82.0827542074107,82.1810337651388,82.2792803442122,
82.3775234272507,82.4792206158929,82.5776050293117,82.6809586055656,82.7843121818195,
82.8829103068232,82.9813680895999,83.0815906573726,83.1798702151008,83.2781167941742,
83.3763598772127,83.4780570658549,83.5764414792737,83.6797950555275,83.7831486317814,
83.8817467567851,83.9802045395618,84.0804271073345,84.1787066650627,84.2769532441361,
84.3751963271746,84.4768935158168,84.5752779292356,84.6786315054894,84.7819850817433,
84.8230016469246),.UNSPECIFIED.);
#556=B_SPLINE_CURVE_WITH_KNOTS('',3,(#55794,#55795,#55796,#55797,#55798,
#55799),.UNSPECIFIED.,.F.,.F.,(4,1,1,4),(84.8230070319842,85.7808215317051,
86.779657981667,87.049742935369),.UNSPECIFIED.);
#557=B_SPLINE_CURVE_WITH_KNOTS('',3,(#55801,#55802,#55803,#55804,#55805,
#55806,#55807,#55808,#55809,#55810,#55811,#55812,#55813,#55814,#55815,#55816,
#55817,#55818,#55819,#55820,#55821,#55822,#55823,#55824,#55825,#55826,#55827,
#55828,#55829,#55830,#55831,#55832,#55833,#55834,#55835,#55836,#55837,#55838,
#55839,#55840,#55841,#55842,#55843,#55844,#55845,#55846,#55847,#55848,#55849,
#55850,#55851,#55852,#55853,#55854,#55855,#55856,#55857,#55858,#55859,#55860,
#55861,#55862,#55863,#55864,#55865,#55866,#55867,#55868,#55869,#55870),
 .UNSPECIFIED.,.F.,.F.,(4,3,3,3,3,3,3,3,3,3,3,3,3,3,3,3,3,3,3,3,3,3,3,4),
(84.8230016472006,84.9261861619504,85.0296647966981,85.1332945907092,85.2372126194224,
85.3160147991856,85.4146129241893,85.513070706966,85.6132932747387,85.7115728324668,
85.8098194115402,85.9080624945786,86.0097596832208,86.1081440966396,86.2114976728935,
86.3148512491474,86.4134243290378,86.5118681332248,86.6102123732649,86.7084866565461,
86.8067399239172,86.9049803913524,87.0032727094652,87.0482730730921),
 .UNSPECIFIED.);
#558=B_SPLINE_CURVE_WITH_KNOTS('',3,(#55871,#55872,#55873,#55874,#55875,
#55876,#55877,#55878,#55879,#55880,#55881,#55882,#55883,#55884,#55885,#55886,
#55887,#55888,#55889,#55890,#55891,#55892,#55893,#55894,#55895,#55896,#55897,
#55898,#55899,#55900,#55901,#55902,#55903,#55904,#55905,#55906,#55907,#55908,
#55909,#55910,#55911,#55912,#55913,#55914,#55915,#55916,#55917,#55918,#55919,
#55920,#55921,#55922,#55923,#55924,#55925,#55926,#55927,#55928,#55929,#55930,
#55931,#55932,#55933,#55934,#55935,#55936,#55937,#55938,#55939,#55940,#55941,
#55942,#55943,#55944,#55945,#55946,#55947,#55948,#55949,#55950,#55951,#55952,
#55953,#55954,#55955,#55956,#55957,#55958,#55959,#55960,#55961,#55962,#55963,
#55964,#55965,#55966,#55967,#55968,#55969,#55970,#55971,#55972,#55973,#55974,
#55975,#55976,#55977,#55978,#55979,#55980,#55981,#55982,#55983,#55984,#55985,
#55986,#55987,#55988,#55989,#55990,#55991,#55992,#55993,#55994),
 .UNSPECIFIED.,.F.,.F.,(4,3,3,3,3,3,3,3,3,3,3,3,3,3,3,3,3,3,3,3,3,3,3,3,
3,3,3,3,3,3,3,3,3,3,3,3,3,3,3,3,3,4),(80.7658264836951,80.8640676560909,
80.9623198605447,81.06067701958,81.1590905825019,81.2576716402341,81.3206689993381,
81.4192671243418,81.5177249071184,81.6179474748911,81.7162270326193,81.8144736116926,
81.9127166947313,82.0144138833734,82.1127982967922,82.2161518730461,82.3195054492999,
82.4181035743036,82.5165613570801,82.6167839248528,82.7150634825809,82.8133100616544,
82.9115531446928,83.0132503333351,83.1116347467539,83.2149883230078,83.3183418992618,
83.4169400242654,83.5153978070421,83.6156203748148,83.7138999325429,83.8121465116161,
83.9103895946545,84.0120867832968,84.1104711967157,84.2138247729697,84.3171783492237,
84.4205578302506,84.5236543867486,84.626583481318,84.7292989065995,84.8230016469246),
 .UNSPECIFIED.);
#559=B_SPLINE_CURVE_WITH_KNOTS('',3,(#56000,#56001,#56002,#56003,#56004,
#56005,#56006,#56007),.UNSPECIFIED.,.F.,.F.,(4,1,1,1,1,4),(74.4816441310534,
74.7936205821245,75.7924570320864,76.7912934820483,77.7901299320101,78.539816339745),
 .UNSPECIFIED.);
#560=B_SPLINE_CURVE_WITH_KNOTS('',3,(#56008,#56009,#56010,#56011,#56012,
#56013,#56014,#56015,#56016,#56017,#56018,#56019,#56020,#56021,#56022,#56023,
#56024,#56025,#56026,#56027,#56028,#56029,#56030,#56031,#56032,#56033,#56034,
#56035,#56036,#56037,#56038,#56039,#56040,#56041,#56042,#56043,#56044,#56045,
#56046,#56047,#56048,#56049,#56050,#56051,#56052,#56053,#56054,#56055,#56056,
#56057,#56058,#56059,#56060,#56061,#56062,#56063,#56064,#56065,#56066,#56067,
#56068,#56069,#56070,#56071,#56072,#56073,#56074),.UNSPECIFIED.,.F.,.F.,
(4,3,3,3,3,3,3,3,3,3,3,3,3,3,3,3,3,3,3,3,3,3,4),(78.5398164398193,78.6677108218625,
78.788966381972,78.8875645069757,78.9860222897523,79.086244857525,79.1845244152531,
79.2827709943266,79.3810140773651,79.4827112660073,79.5810956794261,79.68444925568,
79.7878028319339,79.8864023576698,79.9848611556883,80.0832042043514,80.1814836418338,
80.2797289912676,80.3779697355311,80.4762993937773,80.5746716764715,80.6732109328401,
80.7655329655535),.UNSPECIFIED.);
#561=B_SPLINE_CURVE_WITH_KNOTS('',3,(#56076,#56077,#56078,#56079,#56080,
#56081,#56082,#56083,#56084,#56085,#56086,#56087,#56088,#56089,#56090,#56091,
#56092,#56093,#56094,#56095,#56096,#56097,#56098,#56099,#56100,#56101,#56102,
#56103,#56104,#56105,#56106,#56107,#56108,#56109,#56110,#56111,#56112,#56113,
#56114,#56115,#56116,#56117,#56118,#56119,#56120,#56121,#56122,#56123,#56124,
#56125,#56126,#56127,#56128,#56129,#56130,#56131,#56132,#56133,#56134,#56135,
#56136,#56137,#56138,#56139,#56140,#56141,#56142,#56143,#56144,#56145),
 .UNSPECIFIED.,.F.,.F.,(4,3,3,3,3,3,3,3,3,3,3,3,3,3,3,3,3,3,3,3,3,3,3,4),
(78.539816339745,78.6377138097037,78.7346673304386,78.8315786913981,78.9284788661295,
79.0271081744507,79.1241353185129,79.2235657089636,79.3229960994143,79.421594224418,
79.5200520071949,79.6202745749675,79.7185541326957,79.816800711769,79.9150437948074,
80.0167409834496,80.1151253968684,80.2184789731223,80.3218325493762,80.4204382921282,
80.518879231313,80.6172249291312,80.7155010605349,80.7658264836951),
 .UNSPECIFIED.);
#562=B_SPLINE_CURVE_WITH_KNOTS('',3,(#56146,#56147,#56148,#56149,#56150,
#56151,#56152,#56153),.UNSPECIFIED.,.F.,.F.,(4,1,1,1,1,4),(74.4832630646979,
75.3276502995668,76.3264867495287,77.3253231994906,78.3241596494524,78.539816339745),
 .UNSPECIFIED.);
#563=B_SPLINE_CURVE_WITH_KNOTS('',3,(#56159,#56160,#56161,#56162,#56163,
#56164,#56165,#56166,#56167,#56168,#56169,#56170,#56171,#56172,#56173,#56174,
#56175,#56176,#56177,#56178,#56179,#56180,#56181,#56182,#56183,#56184,#56185,
#56186,#56187,#56188,#56189,#56190,#56191,#56192,#56193,#56194,#56195,#56196,
#56197,#56198,#56199,#56200,#56201,#56202,#56203,#56204,#56205,#56206,#56207,
#56208,#56209,#56210,#56211,#56212,#56213,#56214,#56215,#56216,#56217,#56218,
#56219,#56220,#56221,#56222,#56223,#56224,#56225,#56226,#56227,#56228,#56229,
#56230,#56231,#56232,#56233,#56234,#56235,#56236,#56237,#56238,#56239,#56240,
#56241,#56242,#56243,#56244,#56245,#56246,#56247,#56248,#56249,#56250,#56251,
#56252,#56253,#56254,#56255,#56256,#56257,#56258,#56259,#56260,#56261,#56262,
#56263,#56264,#56265,#56266,#56267,#56268,#56269,#56270,#56271,#56272,#56273,
#56274,#56275,#56276,#56277,#56278,#56279,#56280,#56281,#56282),
 .UNSPECIFIED.,.F.,.F.,(4,3,3,3,3,3,3,3,3,3,3,3,3,3,3,3,3,3,3,3,3,3,3,3,
3,3,3,3,3,3,3,3,3,3,3,3,3,3,3,3,3,4),(68.1995885964076,68.297834762989,
68.3960781129469,68.4972090552985,68.5955944658001,68.6980981740767,68.8006018823533,
68.899200007357,68.9976577901338,69.0978803579064,69.1961599156345,69.2944064947077,
69.3926495777462,69.4943467663884,69.5927311798072,69.6960847560611,69.7994383323151,
69.8980364573188,69.9964942400956,70.0967168078682,70.1949963655964,70.2932429446698,
70.3914860277084,70.4931832163505,70.5915676297693,70.6949212060232,70.798274782277,
70.8968729072806,70.9953306900575,71.0955532578301,71.1938328155582,71.2920793946317,
71.39032247767,71.4920196663122,71.590404079731,71.693757655985,71.7971112322389,
71.902834090551,72.0081993817376,72.1133399321502,72.2181701837246,72.2566308185778),
 .UNSPECIFIED.);
#564=B_SPLINE_CURVE_WITH_KNOTS('',3,(#56283,#56284,#56285,#56286,#56287,
#56288),.UNSPECIFIED.,.F.,.F.,(4,1,1,4),(72.2566310325654,72.7959476822008,
73.7947841321626,74.4816441310534),.UNSPECIFIED.);
#565=B_SPLINE_CURVE_WITH_KNOTS('',3,(#56290,#56291,#56292,#56293,#56294,
#56295,#56296),.UNSPECIFIED.,.F.,.F.,(4,1,1,1,4),(72.2566310325654,72.3311409496812,
73.3299773996431,74.3288138496049,74.4832630646979),.UNSPECIFIED.);
#566=B_SPLINE_CURVE_WITH_KNOTS('',3,(#56297,#56298,#56299,#56300,#56301,
#56302,#56303,#56304,#56305,#56306,#56307,#56308,#56309,#56310,#56311,#56312,
#56313,#56314,#56315,#56316,#56317,#56318,#56319,#56320,#56321,#56322,#56323,
#56324,#56325,#56326,#56327,#56328,#56329,#56330,#56331,#56332,#56333,#56334,
#56335,#56336,#56337,#56338,#56339,#56340,#56341,#56342,#56343,#56344,#56345,
#56346,#56347,#56348,#56349,#56350,#56351,#56352,#56353,#56354,#56355,#56356,
#56357,#56358,#56359,#56360,#56361,#56362,#56363,#56364,#56365,#56366,#56367,
#56368,#56369,#56370,#56371,#56372,#56373,#56374,#56375,#56376,#56377,#56378,
#56379,#56380,#56381,#56382,#56383,#56384,#56385,#56386,#56387,#56388,#56389,
#56390,#56391,#56392,#56393,#56394,#56395,#56396,#56397,#56398,#56399,#56400,
#56401,#56402,#56403,#56404,#56405,#56406,#56407,#56408,#56409,#56410,#56411,
#56412,#56413,#56414,#56415,#56416,#56417,#56418,#56419,#56420,#56421,#56422,
#56423),.UNSPECIFIED.,.F.,.F.,(4,3,3,3,3,3,3,3,3,3,3,3,3,3,3,3,3,3,3,3,
3,3,3,3,3,3,3,3,3,3,3,3,3,3,3,3,3,3,3,3,3,3,4),(68.1987515107913,68.2973434681129,
68.3357951498337,68.4343932748374,68.5328510576141,68.6330736253868,68.7313531831149,
68.8295997621883,68.9278428452268,69.029540033869,69.1279244472878,69.2312780235417,
69.3346315997956,69.4332297247993,69.531687507576,69.6319100753487,69.7301896330768,
69.8284362121502,69.9266792951887,70.0283764838309,70.1267608972497,70.2301144735035,
70.3334680497574,70.4320661747611,70.5305239575379,70.6307465253105,70.7290260830387,
70.8272726621121,70.9255157451506,71.0272129337928,71.1255973472116,71.2289509234654,
71.3323044997193,71.4298807240688,71.527317634942,71.6246428433669,71.7219081150619,
71.8191441424516,71.9163815796695,72.013708783522,72.1110862397604,72.208614546431,
72.2566310325654),.UNSPECIFIED.);
#567=B_SPLINE_CURVE_WITH_KNOTS('',3,(#56429,#56430,#56431,#56432,#56433,
#56434,#56435,#56436),.UNSPECIFIED.,.F.,.F.,(4,1,1,1,1,4),(61.9167164933236,
62.807583182582,63.8064196325439,64.8052560825058,65.8040925324676,65.9734457253857),
 .UNSPECIFIED.);
#568=B_SPLINE_CURVE_WITH_KNOTS('',3,(#56437,#56438,#56439,#56440,#56441,
#56442,#56443,#56444,#56445,#56446,#56447,#56448,#56449,#56450,#56451,#56452,
#56453,#56454,#56455,#56456,#56457,#56458,#56459,#56460,#56461,#56462,#56463,
#56464,#56465,#56466,#56467,#56468,#56469,#56470,#56471,#56472,#56473,#56474,
#56475,#56476,#56477,#56478,#56479,#56480,#56481,#56482,#56483,#56484,#56485,
#56486,#56487,#56488,#56489,#56490,#56491,#56492,#56493,#56494,#56495,#56496,
#56497,#56498,#56499,#56500,#56501,#56502,#56503,#56504,#56505,#56506),
 .UNSPECIFIED.,.F.,.F.,(4,3,3,3,3,3,3,3,3,3,3,3,3,3,3,3,3,3,3,3,3,3,3,4),
(65.9734457253857,66.0704340596178,66.1673127975358,66.264132888756,66.360925426791,
66.4577214670338,66.5546134226801,66.6515579893415,66.7486626585398,66.8029289824295,
66.9015271074332,66.9999848902101,67.1002074579828,67.198487015711,67.2967335947843,
67.3949766778228,67.496673866465,67.5950582798838,67.6984118561376,67.8017654323914,
67.9012212233955,67.9996662412379,68.0996274188227,68.1995885964076),
 .UNSPECIFIED.);
#569=B_SPLINE_CURVE_WITH_KNOTS('',3,(#56508,#56509,#56510,#56511,#56512,
#56513,#56514,#56515,#56516,#56517,#56518,#56519,#56520,#56521,#56522,#56523,
#56524,#56525,#56526,#56527,#56528,#56529,#56530,#56531,#56532,#56533,#56534,
#56535,#56536,#56537,#56538,#56539,#56540,#56541,#56542,#56543,#56544,#56545,
#56546,#56547,#56548,#56549,#56550,#56551,#56552,#56553,#56554,#56555,#56556,
#56557,#56558,#56559,#56560,#56561,#56562,#56563,#56564,#56565,#56566,#56567,
#56568,#56569,#56570,#56571,#56572,#56573,#56574,#56575,#56576,#56577),
 .UNSPECIFIED.,.F.,.F.,(4,3,3,3,3,3,3,3,3,3,3,3,3,3,3,3,3,3,3,3,3,3,3,4),
(65.9734457256204,66.0848798050736,66.1968635637033,66.3094957826818,66.3381222499099,
66.4367203749136,66.5351781576903,66.635400725463,66.7336802831912,66.8319268622646,
66.930169945303,67.0318671339452,67.130251547364,67.2336051236179,67.3369586998718,
67.4355663370596,67.5340045943448,67.6323466348067,67.7306220560095,67.828860384381,
67.9271329658743,68.0254205103658,68.123818393505,68.1987515107913),
 .UNSPECIFIED.);
#570=B_SPLINE_CURVE_WITH_KNOTS('',3,(#56578,#56579,#56580,#56581,#56582,
#56583,#56584,#56585,#56586,#56587,#56588,#56589,#56590,#56591,#56592,#56593,
#56594,#56595,#56596,#56597,#56598,#56599,#56600,#56601,#56602,#56603,#56604,
#56605,#56606,#56607,#56608,#56609,#56610,#56611,#56612,#56613,#56614,#56615,
#56616,#56617,#56618,#56619,#56620,#56621,#56622,#56623,#56624,#56625,#56626,
#56627,#56628,#56629,#56630,#56631,#56632,#56633,#56634,#56635,#56636,#56637,
#56638,#56639,#56640,#56641,#56642,#56643,#56644,#56645,#56646,#56647,#56648,
#56649,#56650,#56651,#56652,#56653,#56654,#56655,#56656,#56657,#56658,#56659,
#56660,#56661,#56662,#56663,#56664,#56665,#56666,#56667,#56668,#56669,#56670,
#56671,#56672,#56673,#56674,#56675,#56676,#56677,#56678,#56679,#56680,#56681,
#56682,#56683,#56684,#56685,#56686,#56687,#56688,#56689,#56690,#56691,#56692,
#56693,#56694,#56695,#56696,#56697,#56698,#56699,#56700,#56701,#56702,#56703,
#56704),.UNSPECIFIED.,.F.,.F.,(4,3,3,3,3,3,3,3,3,3,3,3,3,3,3,3,3,3,3,3,
3,3,3,3,3,3,3,3,3,3,3,3,3,3,3,3,3,3,3,3,3,3,4),(61.9158792705717,62.0141406127527,
62.1125120200468,62.2109478399191,62.3095423749078,62.3427764500624,62.4413745750661,
62.539832357843,62.6400549256157,62.7383344833438,62.8365810624172,62.9348241454557,
63.0365213340979,63.1349057475167,63.2382593237705,63.3416129000243,63.440211025028,
63.5386688078047,63.6388913755774,63.7371709333055,63.835417512379,63.9336605954174,
64.0353577840596,64.1337421974785,64.2370957737323,64.3404493499862,64.4390474749899,
64.5375052577665,64.6377278255392,64.7360073832674,64.8342539623408,64.9324970453791,
65.0341942340214,65.13257864744,65.2359322236941,65.3392857999481,65.4384637976085,
65.53749807745,65.6364173808604,65.7352455972606,65.8340208922139,65.932784900221,
65.9734457253857),.UNSPECIFIED.);
#571=B_SPLINE_CURVE_WITH_KNOTS('',3,(#56710,#56711,#56712,#56713,#56714,
#56715,#56716,#56717,#56718,#56719,#56720,#56721,#56722,#56723,#56724,#56725,
#56726,#56727,#56728,#56729,#56730,#56731,#56732,#56733,#56734,#56735,#56736,
#56737,#56738,#56739,#56740,#56741,#56742,#56743,#56744,#56745,#56746,#56747,
#56748,#56749,#56750,#56751,#56752,#56753,#56754,#56755,#56756,#56757,#56758,
#56759,#56760,#56761,#56762,#56763,#56764,#56765,#56766,#56767,#56768,#56769,
#56770,#56771,#56772,#56773,#56774,#56775,#56776,#56777,#56778,#56779,#56780,
#56781,#56782,#56783,#56784,#56785,#56786,#56787,#56788,#56789,#56790,#56791,
#56792,#56793,#56794,#56795,#56796,#56797,#56798,#56799,#56800,#56801,#56802,
#56803,#56804,#56805,#56806,#56807,#56808,#56809,#56810,#56811,#56812,#56813,
#56814,#56815,#56816,#56817,#56818,#56819,#56820,#56821,#56822,#56823,#56824,
#56825,#56826,#56827,#56828,#56829,#56830,#56831,#56832,#56833),
 .UNSPECIFIED.,.F.,.F.,(4,3,3,3,3,3,3,3,3,3,3,3,3,3,3,3,3,3,3,3,3,3,3,3,
3,3,3,3,3,3,3,3,3,3,3,3,3,3,3,3,3,4),(55.6323252053611,55.7308982696372,
55.8157280328489,55.9143261578526,56.0127839406294,56.1130065084021,56.2112860661302,
56.3095326452036,56.4077757282421,56.5094729168843,56.6078573303031,56.7112109065569,
56.8145644828108,56.9131626078145,57.0116203905912,57.1118429583639,57.210122516092,
57.3083690951654,57.4066121782039,57.5083093668461,57.6066937802649,57.7100473565188,
57.8134009327727,57.9119990577764,58.0104568405531,58.1106794083258,58.2089589660539,
58.3072055451273,58.4054486281658,58.5071458168079,58.6055302302267,58.7088838064806,
58.8122373827345,58.9094791608007,59.0070768179764,59.1040671063403,59.2009981633324,
59.2979009849176,59.3959908432397,59.4929780422904,59.5916192302483,59.6902604182062),
 .UNSPECIFIED.);
#572=B_SPLINE_CURVE_WITH_KNOTS('',3,(#56834,#56835,#56836,#56837,#56838,
#56839,#56840),.UNSPECIFIED.,.F.,.F.,(4,1,1,1,4),(59.6902604182062,59.8110738326964,
60.8099102826583,61.8087467326202,61.9167164933236),.UNSPECIFIED.);
#573=B_SPLINE_CURVE_WITH_KNOTS('',3,(#56842,#56843,#56844,#56845,#56846,
#56847,#56848,#56849,#56850,#56851,#56852,#56853,#56854,#56855,#56856,#56857,
#56858,#56859,#56860,#56861,#56862,#56863,#56864,#56865,#56866,#56867,#56868,
#56869,#56870,#56871,#56872,#56873,#56874,#56875,#56876,#56877,#56878,#56879,
#56880,#56881,#56882,#56883,#56884,#56885,#56886,#56887,#56888,#56889,#56890,
#56891,#56892,#56893,#56894,#56895,#56896,#56897,#56898,#56899,#56900,#56901,
#56902,#56903,#56904,#56905,#56906,#56907,#56908,#56909,#56910,#56911),
 .UNSPECIFIED.,.F.,.F.,(4,3,3,3,3,3,3,3,3,3,3,3,3,3,3,3,3,3,3,3,3,3,3,4),
(59.6902604182062,59.788634173056,59.886998581597,59.9853827919993,60.0838846667643,
60.1824499292137,60.2811933482975,60.3451035501387,60.4437016751424,60.542159457919,
60.6423820256917,60.7406615834199,60.8389081624932,60.9371512455317,61.0388484341739,
61.1372328475927,61.2405864238466,61.3439400001006,61.4425291322751,61.5409847704255,
61.639327281874,61.7376024228517,61.8358589218597,61.9158792705717),
 .UNSPECIFIED.);
#574=B_SPLINE_CURVE_WITH_KNOTS('',3,(#56912,#56913,#56914,#56915,#56916,
#56917,#56918,#56919,#56920,#56921,#56922,#56923,#56924,#56925,#56926,#56927,
#56928,#56929,#56930,#56931,#56932,#56933,#56934,#56935,#56936,#56937,#56938,
#56939,#56940,#56941,#56942,#56943,#56944,#56945,#56946,#56947,#56948,#56949,
#56950,#56951,#56952,#56953,#56954,#56955,#56956,#56957,#56958,#56959,#56960,
#56961,#56962,#56963,#56964,#56965,#56966,#56967,#56968,#56969,#56970,#56971,
#56972,#56973,#56974,#56975,#56976,#56977,#56978,#56979,#56980,#56981,#56982,
#56983,#56984,#56985,#56986,#56987,#56988,#56989,#56990,#56991,#56992,#56993,
#56994,#56995,#56996,#56997,#56998,#56999,#57000,#57001,#57002,#57003,#57004,
#57005,#57006,#57007,#57008,#57009,#57010,#57011,#57012,#57013,#57014,#57015,
#57016,#57017,#57018,#57019,#57020,#57021,#57022,#57023,#57024,#57025,#57026,
#57027,#57028,#57029,#57030,#57031,#57032,#57033,#57034,#57035),
 .UNSPECIFIED.,.F.,.F.,(4,3,3,3,3,3,3,3,3,3,3,3,3,3,3,3,3,3,3,3,3,3,3,3,
3,3,3,3,3,3,3,3,3,3,3,3,3,3,3,3,3,4),(55.633462551168,55.73174959566,55.8299992392,
55.9282409685686,56.0265042540639,56.1248785008508,56.2233186112086,56.3219159061656,
56.3497577502912,56.4483558752949,56.5468136580715,56.6470362258442,56.7453157835724,
56.8435623626458,56.9418054456843,57.0435026343265,57.1418870477454,57.2452406239993,
57.3485942002531,57.4471923252568,57.5456501080335,57.6458726758062,57.7441522335343,
57.8423988126077,57.9406418956462,58.0423390842884,58.1407234977072,58.244077073961,
58.3474306502149,58.4460287752184,58.5444865579953,58.644709125768,58.7429886834962,
58.8412352625695,58.9394783456081,59.0411755342503,59.1395599476691,59.242913523923,
59.3462671001768,59.4608829140295,59.5755716660044,59.6902604179793),
 .UNSPECIFIED.);
#575=B_SPLINE_CURVE_WITH_KNOTS('',3,(#57041,#57042,#57043,#57044,#57045,
#57046,#57047,#57048),.UNSPECIFIED.,.F.,.F.,(4,1,1,1,1,4),(49.3495871987639,
49.8227093330777,50.8215457830395,51.8203822330014,52.8192186829633,53.4070751110266),
 .UNSPECIFIED.);
#576=B_SPLINE_CURVE_WITH_KNOTS('',3,(#57049,#57050,#57051,#57052,#57053,
#57054,#57055,#57056,#57057,#57058,#57059,#57060,#57061,#57062,#57063,#57064,
#57065,#57066,#57067,#57068,#57069,#57070,#57071,#57072,#57073,#57074,#57075,
#57076,#57077,#57078,#57079,#57080,#57081,#57082,#57083,#57084,#57085,#57086,
#57087,#57088,#57089,#57090,#57091,#57092,#57093,#57094,#57095,#57096,#57097,
#57098,#57099,#57100,#57101,#57102,#57103,#57104,#57105,#57106,#57107,#57108,
#57109,#57110,#57111,#57112,#57113,#57114,#57115,#57116,#57117,#57118),
 .UNSPECIFIED.,.F.,.F.,(4,3,3,3,3,3,3,3,3,3,3,3,3,3,3,3,3,3,3,3,3,3,3,4),
(53.4070755243676,53.5149520672777,53.623163861073,53.7318758460237,53.8180551329252,
53.9166532579289,54.0151110407056,54.1153336084783,54.2136131662064,54.3118597452797,
54.4101028283182,54.5118000169604,54.6101844303792,54.7135380066331,54.816891582887,
54.9188207856963,55.0172568628781,55.1155965182368,55.2138693497382,55.3121048835941,
55.4103643250343,55.5086391377704,55.6069975900418,55.6323252053611),
 .UNSPECIFIED.);
#577=B_SPLINE_CURVE_WITH_KNOTS('',3,(#57120,#57121,#57122,#57123,#57124,
#57125,#57126,#57127,#57128,#57129,#57130,#57131,#57132,#57133,#57134,#57135,
#57136,#57137,#57138,#57139,#57140,#57141,#57142,#57143,#57144,#57145,#57146,
#57147,#57148,#57149,#57150,#57151,#57152,#57153,#57154,#57155,#57156,#57157,
#57158,#57159,#57160,#57161,#57162,#57163,#57164,#57165,#57166,#57167,#57168,
#57169,#57170,#57171,#57172,#57173,#57174,#57175,#57176,#57177,#57178,#57179,
#57180,#57181,#57182,#57183,#57184,#57185,#57186,#57187,#57188,#57189),
 .UNSPECIFIED.,.F.,.F.,(4,3,3,3,3,3,3,3,3,3,3,3,3,3,3,3,3,3,3,3,3,3,3,4),
(53.4070751110266,53.5048543854907,53.6024983707772,53.7000367768846,53.7975186210126,
53.8949743677963,53.9924344477706,54.0899931990358,54.1876041339868,54.2853815723763,
54.3520848503674,54.4506829753711,54.5491407581476,54.6493633259203,54.7476428836485,
54.8458894627219,54.9441325457605,55.0458297344027,55.1442141478214,55.2475677240754,
55.3509213003293,55.449511235452,55.5479503969111,55.633462551168),
 .UNSPECIFIED.);
#578=B_SPLINE_CURVE_WITH_KNOTS('',3,(#57190,#57191,#57192,#57193,#57194,
#57195,#57196,#57197,#57198),.UNSPECIFIED.,.F.,.F.,(4,1,1,1,1,1,4),(49.349677120857,
49.3579026005581,50.3567390505199,51.3555755004818,52.3544119504437,53.3532484004056,
53.4070751110266),.UNSPECIFIED.);
#579=B_SPLINE_CURVE_WITH_KNOTS('',3,(#57204,#57205,#57206,#57207,#57208,
#57209,#57210,#57211,#57212,#57213,#57214,#57215,#57216,#57217,#57218,#57219,
#57220,#57221,#57222,#57223,#57224,#57225,#57226,#57227,#57228,#57229,#57230,
#57231,#57232,#57233,#57234,#57235,#57236,#57237,#57238,#57239,#57240,#57241,
#57242,#57243,#57244,#57245,#57246,#57247,#57248,#57249,#57250,#57251,#57252,
#57253,#57254,#57255,#57256,#57257,#57258,#57259,#57260,#57261,#57262,#57263,
#57264,#57265,#57266,#57267,#57268,#57269,#57270,#57271,#57272,#57273,#57274,
#57275,#57276,#57277,#57278,#57279,#57280,#57281,#57282,#57283,#57284,#57285,
#57286,#57287,#57288,#57289,#57290,#57291,#57292,#57293,#57294,#57295,#57296,
#57297,#57298,#57299,#57300,#57301,#57302,#57303,#57304,#57305,#57306,#57307,
#57308,#57309,#57310,#57311,#57312,#57313,#57314,#57315,#57316,#57317,#57318,
#57319,#57320,#57321,#57322,#57323,#57324,#57325,#57326,#57327),
 .UNSPECIFIED.,.F.,.F.,(4,3,3,3,3,3,3,3,3,3,3,3,3,3,3,3,3,3,3,3,3,3,3,3,
3,3,3,3,3,3,3,3,3,3,3,3,3,3,3,3,3,4),(43.0671358462258,43.1654506957331,
43.2637142592363,43.3619560404535,43.4602055141326,43.5585579558209,43.6569638005109,
43.7555405747165,43.8296906333064,43.9282887583114,44.0267465410897,44.126969108862,
44.2252486665916,44.3234952456665,44.4217383287065,44.523435517347,44.6218199307672,
44.7251735070178,44.8285270832683,44.9271252082715,45.025582991048,45.1258055588207,
45.2240851165484,45.3223316956214,45.4205747786595,45.5222719673022,45.6206563807206,
45.7240099569754,45.8273635332302,45.9259616582337,46.0244194410101,46.1246420087828,
46.2229215665108,46.3211681455839,46.4194112286225,46.5211084172648,46.6194928306836,
46.7228464069378,46.826199983192,46.9466622822351,47.0654828012647,47.1238896269613),
 .UNSPECIFIED.);
#580=B_SPLINE_CURVE_WITH_KNOTS('',3,(#57328,#57329,#57330,#57331,#57332,
#57333),.UNSPECIFIED.,.F.,.F.,(4,1,1,4),(47.123889803847,47.8250364331539,
48.8238728831158,49.3495871987639),.UNSPECIFIED.);
#581=B_SPLINE_CURVE_WITH_KNOTS('',3,(#57335,#57336,#57337,#57338,#57339,
#57340),.UNSPECIFIED.,.F.,.F.,(4,1,1,4),(47.1238901028405,47.3602297006343,
48.3590661505962,49.349677120857),.UNSPECIFIED.);
#582=B_SPLINE_CURVE_WITH_KNOTS('',3,(#57341,#57342,#57343,#57344,#57345,
#57346,#57347,#57348,#57349,#57350,#57351,#57352,#57353,#57354,#57355,#57356,
#57357,#57358,#57359,#57360,#57361,#57362,#57363,#57364,#57365,#57366,#57367,
#57368,#57369,#57370,#57371,#57372,#57373,#57374,#57375,#57376,#57377,#57378,
#57379,#57380,#57381,#57382,#57383,#57384,#57385,#57386,#57387,#57388,#57389,
#57390,#57391,#57392,#57393,#57394,#57395,#57396,#57397,#57398,#57399,#57400,
#57401,#57402,#57403,#57404,#57405,#57406,#57407,#57408,#57409,#57410,#57411,
#57412,#57413,#57414,#57415,#57416,#57417,#57418,#57419,#57420,#57421,#57422,
#57423,#57424,#57425,#57426,#57427,#57428,#57429,#57430,#57431,#57432,#57433,
#57434,#57435,#57436,#57437,#57438,#57439,#57440,#57441,#57442,#57443,#57444,
#57445,#57446,#57447,#57448,#57449,#57450,#57451,#57452,#57453,#57454,#57455,
#57456,#57457,#57458,#57459,#57460,#57461,#57462,#57463,#57464),
 .UNSPECIFIED.,.F.,.F.,(4,3,3,3,3,3,3,3,3,3,3,3,3,3,3,3,3,3,3,3,3,3,3,3,
3,3,3,3,3,3,3,3,3,3,3,3,3,3,3,3,3,4),(43.0660207909132,43.1644088987463,
43.2646463997666,43.3648839007868,43.4634820258002,43.5619398085867,43.6621623763569,
43.7604419340952,43.8586885131787,43.9569315962273,44.0586287848577,44.1570131982869,
44.2603667745178,44.3637203507487,44.4623184757497,44.5607762585238,44.6609988262972,
44.7592783840227,44.8575249630933,44.955768046129,45.0574652347744,45.1558496481904,
45.2592032244505,45.3625568007106,45.4611549257133,45.5596127084892,45.6598352762621,
45.758114833989,45.8563614130613,45.9546044960985,46.056301684742,46.1546860981596,
46.258039674416,46.3613932506724,46.4587199838046,46.5559210250953,46.6530274701202,
46.7500702965176,46.8471124553619,46.9441490048062,47.0412721236582,47.123889803847),
 .UNSPECIFIED.);
#583=B_SPLINE_CURVE_WITH_KNOTS('',3,(#57470,#57471,#57472,#57473,#57474,
#57475,#57476,#57477,#57478,#57479,#57480,#57481,#57482,#57483,#57484,#57485,
#57486,#57487,#57488,#57489,#57490,#57491,#57492,#57493,#57494,#57495,#57496,
#57497,#57498,#57499,#57500,#57501,#57502,#57503,#57504,#57505,#57506,#57507,
#57508,#57509,#57510,#57511,#57512,#57513,#57514,#57515,#57516,#57517,#57518,
#57519,#57520,#57521,#57522,#57523,#57524,#57525,#57526,#57527,#57528,#57529,
#57530,#57531,#57532,#57533,#57534,#57535,#57536,#57537,#57538,#57539,#57540,
#57541,#57542,#57543,#57544,#57545,#57546,#57547,#57548,#57549,#57550,#57551,
#57552,#57553,#57554,#57555,#57556,#57557,#57558,#57559,#57560,#57561,#57562,
#57563,#57564,#57565,#57566,#57567,#57568,#57569,#57570,#57571,#57572,#57573,
#57574,#57575,#57576,#57577,#57578,#57579,#57580,#57581,#57582,#57583,#57584,
#57585,#57586,#57587,#57588,#57589,#57590,#57591,#57592,#57593,#57594,#57595,
#57596),.UNSPECIFIED.,.F.,.F.,(4,3,3,3,3,3,3,3,3,3,3,3,3,3,3,3,3,3,3,3,
3,3,3,3,3,3,3,3,3,3,3,3,3,3,3,3,3,3,3,3,3,3,4),(36.7830721337714,36.8378354835733,
36.9364336084865,37.034891391171,37.1351139589665,37.2333935165987,37.3316400955748,
37.429883178515,37.5315803672701,37.6299647805889,37.7333183570621,37.8366719335352,
37.9352700586078,38.0337278414544,38.1339504092097,38.2322299670096,38.3304765461552,
38.4287196292664,38.530416817824,38.6288012313159,38.7321548074064,38.835508383497,
38.9341065084864,39.0325642912487,39.132786859025,39.2310664167387,39.3293129957976,
39.4275560788218,39.5292532674811,39.6276376808857,39.7309912571723,39.8343448334589,
39.9329429584521,40.0314007412181,40.1316233089935,40.2299028667104,40.3281494457725,
40.4263925287994,40.5280897174548,40.6264741308618,40.7298277071413,40.8331812834208,
40.8407044966674),.UNSPECIFIED.);
#584=B_SPLINE_CURVE_WITH_KNOTS('',3,(#57597,#57598,#57599,#57600,#57601,
#57602,#57603,#57604,#57605,#57606,#57607,#57608,#57609,#57610,#57611,#57612,
#57613,#57614,#57615,#57616,#57617,#57618,#57619,#57620,#57621,#57622,#57623,
#57624,#57625,#57626,#57627,#57628,#57629,#57630,#57631,#57632,#57633,#57634,
#57635,#57636,#57637,#57638,#57639,#57640,#57641,#57642,#57643,#57644,#57645,
#57646,#57647,#57648,#57649,#57650,#57651,#57652,#57653,#57654,#57655,#57656,
#57657,#57658,#57659,#57660,#57661,#57662,#57663,#57664,#57665,#57666),
 .UNSPECIFIED.,.F.,.F.,(4,3,3,3,3,3,3,3,3,3,3,3,3,3,3,3,3,3,3,3,3,3,3,4),
(40.8407044969197,40.9391705387199,41.0374964280042,41.1368115911765,41.2349607512895,
41.3330774110131,41.4311912274066,41.5313978539006,41.6296531901077,41.7308354617452,
41.8320177333827,41.9306158583837,42.0290736411578,42.1292962089311,42.2275757666566,
42.3258223457272,42.4240654287629,42.5257626174083,42.6241470308245,42.7275006070845,
42.8308541833445,42.929455918813,43.027905177827,43.0671358462258),
 .UNSPECIFIED.);
#585=B_SPLINE_CURVE_WITH_KNOTS('',3,(#57668,#57669,#57670,#57671,#57672,
#57673,#57674,#57675,#57676,#57677,#57678,#57679,#57680,#57681,#57682,#57683,
#57684,#57685,#57686,#57687,#57688,#57689,#57690,#57691,#57692,#57693,#57694,
#57695,#57696,#57697,#57698,#57699,#57700,#57701,#57702,#57703,#57704,#57705,
#57706,#57707,#57708,#57709,#57710,#57711,#57712,#57713,#57714,#57715,#57716,
#57717,#57718,#57719,#57720,#57721,#57722,#57723,#57724,#57725,#57726,#57727,
#57728,#57729,#57730,#57731,#57732,#57733,#57734,#57735,#57736,#57737),
 .UNSPECIFIED.,.F.,.F.,(4,3,3,3,3,3,3,3,3,3,3,3,3,3,3,3,3,3,3,3,3,3,3,4),
(40.8407044966674,40.9425310419931,41.0487010317106,41.1508691915794,41.2531658485544,
41.3556785603232,41.3672110008631,41.4658091258525,41.5642669086152,41.6644894763914,
41.7627690341051,41.8610156131643,41.9592586961885,42.0609558848476,42.1593402982524,
42.2626938745386,42.3660474508249,42.4646234053299,42.5630692109005,42.6614145831975,
42.7625661351264,42.8608128976382,42.9634168442757,43.0660207909132),
 .UNSPECIFIED.);
#586=B_SPLINE_CURVE_WITH_KNOTS('',3,(#57738,#57739,#57740,#57741,#57742,
#57743,#57744,#57745),.UNSPECIFIED.,.F.,.F.,(4,1,1,1,1,4),(36.7838197989548,
37.3718652010156,38.3707016509774,39.3695381009393,40.3683745509012,40.8407024149584),
 .UNSPECIFIED.);
#587=B_SPLINE_CURVE_WITH_KNOTS('',3,(#57751,#57752,#57753,#57754,#57755,
#57756,#57757,#57758,#57759,#57760,#57761,#57762,#57763,#57764,#57765,#57766,
#57767,#57768,#57769,#57770,#57771,#57772,#57773,#57774,#57775,#57776,#57777,
#57778,#57779,#57780,#57781,#57782,#57783,#57784,#57785,#57786,#57787,#57788,
#57789,#57790,#57791,#57792,#57793,#57794,#57795,#57796,#57797,#57798,#57799,
#57800,#57801,#57802,#57803,#57804,#57805,#57806,#57807,#57808,#57809,#57810,
#57811,#57812,#57813,#57814,#57815,#57816,#57817,#57818,#57819,#57820,#57821,
#57822,#57823,#57824,#57825,#57826,#57827,#57828,#57829,#57830,#57831,#57832,
#57833,#57834,#57835,#57836,#57837,#57838,#57839,#57840,#57841,#57842,#57843,
#57844,#57845,#57846,#57847,#57848,#57849,#57850,#57851,#57852,#57853,#57854,
#57855,#57856,#57857,#57858,#57859,#57860,#57861,#57862,#57863,#57864,#57865,
#57866,#57867,#57868,#57869,#57870,#57871,#57872,#57873,#57874,#57875,#57876,
#57877),.UNSPECIFIED.,.F.,.F.,(4,3,3,3,3,3,3,3,3,3,3,3,3,3,3,3,3,3,3,3,
3,3,3,3,3,3,3,3,3,3,3,3,3,3,3,3,3,3,3,3,3,3,4),(30.4997392209955,30.59810244627,
30.6965256522857,30.7951123625252,30.844816783802,30.9434149029147,31.041872679697,
31.1420952489554,31.240374800478,31.3386213732805,31.4368644499908,31.5385616459341,
31.636946052946,31.7402996433549,31.8436532337639,31.9422513619748,32.040709147999,
32.1409317149648,32.2392112760154,32.3374578584321,32.4357009448303,32.5373981295542,
32.6357825463393,32.7391361150326,32.8424896837258,32.9410878085143,33.0395455910813,
33.1397681589071,33.2380477164402,33.3362942953243,33.4345373781799,33.5362345670568,
33.6346189803102,33.737972556999,33.8413261336877,33.93909739415,34.0367388270534,
34.1342810926871,34.2317547370018,34.3292101035708,34.426655495324,34.5241539308998,
34.5575191894878),.UNSPECIFIED.);
#588=B_SPLINE_CURVE_WITH_KNOTS('',3,(#57878,#57879,#57880,#57881,#57882,
#57883,#57884,#57885,#57886,#57887,#57888,#57889,#57890,#57891,#57892,#57893,
#57894,#57895,#57896,#57897,#57898,#57899,#57900,#57901,#57902,#57903,#57904,
#57905,#57906,#57907,#57908,#57909,#57910,#57911,#57912,#57913,#57914,#57915,
#57916,#57917,#57918,#57919,#57920,#57921,#57922,#57923,#57924,#57925,#57926,
#57927,#57928,#57929,#57930,#57931,#57932,#57933,#57934,#57935,#57936,#57937,
#57938,#57939,#57940,#57941,#57942,#57943,#57944,#57945,#57946,#57947),
 .UNSPECIFIED.,.F.,.F.,(4,3,3,3,3,3,3,3,3,3,3,3,3,3,3,3,3,3,3,3,3,3,3,4),
(34.5575191897594,34.6782345503608,34.8009387396036,34.8401625836495,34.9387607091287,
35.0372184923873,35.1374410600403,35.2357206182623,35.333967197833,35.4322102813716,
35.5339074694315,35.6322918833522,35.7356454584818,35.8389990336114,35.9376008413507,
36.036061306603,36.1344037647034,36.2326817408431,36.3309247589446,36.429162301612,
36.5274785677215,36.6258371036485,36.7243383500844,36.7830721337714),
 .UNSPECIFIED.);
#589=B_SPLINE_CURVE_WITH_KNOTS('',3,(#57949,#57950,#57951,#57952,#57953,
#57954),.UNSPECIFIED.,.F.,.F.,(4,1,1,4),(34.5575241471828,35.3741923010918,
36.3730287510537,36.7838197989548),.UNSPECIFIED.);
#590=B_SPLINE_CURVE_WITH_KNOTS('',3,(#57955,#57956,#57957,#57958,#57959,
#57960,#57961,#57962,#57963,#57964,#57965,#57966,#57967,#57968,#57969,#57970,
#57971,#57972,#57973,#57974,#57975,#57976,#57977,#57978,#57979,#57980,#57981,
#57982,#57983,#57984,#57985,#57986,#57987,#57988,#57989,#57990,#57991,#57992,
#57993,#57994,#57995,#57996,#57997,#57998,#57999,#58000,#58001,#58002,#58003,
#58004,#58005,#58006,#58007,#58008,#58009,#58010,#58011,#58012,#58013,#58014,
#58015,#58016,#58017,#58018,#58019,#58020,#58021,#58022,#58023,#58024,#58025,
#58026,#58027,#58028,#58029,#58030,#58031,#58032,#58033,#58034,#58035,#58036,
#58037,#58038,#58039,#58040,#58041,#58042,#58043,#58044,#58045,#58046,#58047,
#58048,#58049,#58050,#58051,#58052,#58053,#58054,#58055,#58056,#58057,#58058,
#58059,#58060,#58061,#58062,#58063,#58064,#58065,#58066,#58067,#58068,#58069,
#58070,#58071,#58072,#58073,#58074,#58075,#58076,#58077,#58078),
 .UNSPECIFIED.,.F.,.F.,(4,3,3,3,3,3,3,3,3,3,3,3,3,3,3,3,3,3,3,3,3,3,3,3,
3,3,3,3,3,3,3,3,3,3,3,3,3,3,3,3,3,4),(30.5006744577879,30.5991052616483,
30.6974320572743,30.7957024061211,30.893945819764,30.9921917761612,31.0905375611812,
31.1889321228201,31.2875030639315,31.3788465012443,31.4774446472309,31.575902451235,
31.6761250137314,31.7744045931314,31.8726511939953,31.9708942989141,32.0725914619871,
32.1709758972869,32.2743294242465,32.3776829512062,32.4762810765969,32.5747388598271,
32.6749614274947,32.7732409858373,32.871487565584,32.9697306493543,33.0714278373078,
33.1698122515977,33.2731658263829,33.3765194011681,33.4751175203039,33.5735752971096,
33.6737978663622,33.7720774179092,33.8703239907363,33.9685670674716,34.0702642633862,
34.1686486704234,34.2720022607767,34.37535585113,34.5238559809678,34.5575191894878),
 .UNSPECIFIED.);
#591=B_SPLINE_CURVE_WITH_KNOTS('',3,(#58084,#58085,#58086,#58087,#58088,
#58089,#58090,#58091),.UNSPECIFIED.,.F.,.F.,(4,1,1,1,1,4),(24.2176478214031,
24.8517980840308,25.8506345339927,26.8494709839545,27.8483074339164,28.2743284148014),
 .UNSPECIFIED.);
#592=B_SPLINE_CURVE_WITH_KNOTS('',3,(#58092,#58093,#58094,#58095,#58096,
#58097,#58098,#58099,#58100,#58101,#58102,#58103,#58104,#58105,#58106,#58107,
#58108,#58109,#58110,#58111,#58112,#58113,#58114,#58115,#58116,#58117,#58118,
#58119,#58120,#58121,#58122,#58123,#58124,#58125,#58126,#58127,#58128,#58129,
#58130,#58131,#58132,#58133,#58134,#58135,#58136,#58137,#58138,#58139,#58140,
#58141,#58142,#58143,#58144,#58145,#58146,#58147,#58148,#58149,#58150,#58151,
#58152,#58153,#58154,#58155,#58156,#58157,#58158,#58159,#58160,#58161),
 .UNSPECIFIED.,.F.,.F.,(4,3,3,3,3,3,3,3,3,3,3,3,3,3,3,3,3,3,3,3,3,3,3,4),
(28.2743338823082,28.3746245106346,28.4749734038757,28.575488632026,28.6760922702813,
28.7769068624063,28.8471438838783,28.9457420299521,29.0441998340446,29.144422396519,
29.2427019760093,29.340948576964,29.4391916819737,29.5408888449403,29.6392732803313,
29.7426268070858,29.8459803338402,29.9445606477205,30.0430096057643,30.1413569295321,
30.2396381186445,30.3378792535306,30.4361386871608,30.4997392209955),
 .UNSPECIFIED.);
#593=B_SPLINE_CURVE_WITH_KNOTS('',3,(#58163,#58164,#58165,#58166,#58167,
#58168,#58169,#58170,#58171,#58172,#58173,#58174,#58175,#58176,#58177,#58178,
#58179,#58180,#58181,#58182,#58183,#58184,#58185,#58186,#58187,#58188,#58189,
#58190,#58191,#58192,#58193,#58194,#58195,#58196,#58197,#58198,#58199,#58200,
#58201,#58202,#58203,#58204,#58205,#58206,#58207,#58208,#58209,#58210,#58211,
#58212,#58213,#58214,#58215,#58216,#58217,#58218,#58219,#58220,#58221,#58222,
#58223,#58224,#58225,#58226,#58227,#58228,#58229,#58230,#58231,#58232),
 .UNSPECIFIED.,.F.,.F.,(4,3,3,3,3,3,3,3,3,3,3,3,3,3,3,3,3,3,3,3,3,3,3,4),
(28.2743338823082,28.3823371513587,28.4809354100483,28.5793933279209,28.6796158620959,
28.7778955573906,28.876142274651,28.9743854963144,29.0760825225659,29.1744670742836,
29.2778203378021,29.3811736013206,29.47977174272,29.5782295425626,29.6784521061526,
29.7767316824779,29.8749782806812,29.9732213833591,30.07491855034,30.173302984478,
30.2766565178802,30.3800100512825,30.4786103666735,30.5006744577879),
 .UNSPECIFIED.);
#594=B_SPLINE_CURVE_WITH_KNOTS('',3,(#58233,#58234,#58235,#58236,#58237,
#58238,#58239,#58240,#58241,#58242,#58243,#58244,#58245,#58246,#58247,#58248,
#58249,#58250,#58251,#58252,#58253,#58254,#58255,#58256,#58257,#58258,#58259,
#58260,#58261,#58262,#58263,#58264,#58265,#58266,#58267,#58268,#58269,#58270,
#58271,#58272,#58273,#58274,#58275,#58276,#58277,#58278,#58279,#58280,#58281,
#58282,#58283,#58284,#58285,#58286,#58287,#58288,#58289,#58290,#58291,#58292,
#58293,#58294,#58295,#58296,#58297,#58298,#58299,#58300,#58301,#58302,#58303,
#58304,#58305,#58306,#58307,#58308,#58309,#58310,#58311,#58312,#58313,#58314,
#58315,#58316,#58317,#58318,#58319,#58320,#58321,#58322,#58323,#58324,#58325,
#58326,#58327,#58328,#58329,#58330,#58331,#58332,#58333,#58334,#58335,#58336,
#58337,#58338,#58339,#58340,#58341,#58342,#58343,#58344,#58345,#58346,#58347,
#58348,#58349,#58350,#58351,#58352,#58353,#58354,#58355,#58356,#58357,#58358,
#58359),.UNSPECIFIED.,.F.,.F.,(4,3,3,3,3,3,3,3,3,3,3,3,3,3,3,3,3,3,3,3,
3,3,3,3,3,3,3,3,3,3,3,3,3,3,3,3,3,3,3,3,3,3,4),(24.2164091264089,24.3149891732794,
24.3869913515112,24.4855869800636,24.5840422282253,24.6842654248812,24.7825423726193,
24.8807863192412,24.9790267507949,25.0807270134645,25.1791087548177,25.2824682781454,
25.3858278014731,25.4844267451928,25.5828853541422,25.6831077163038,25.7813881124234,
25.8796355326055,25.9778794583543,26.0795756566245,26.1779609081003,26.2813125797677,
26.384664251435,26.4832625888131,26.5817205900565,26.681943103974,26.780222893609,
26.8784697091132,26.9767130328096,27.0784099499564,27.1767946121896,27.2801476567932,
27.3835007013968,27.4808124356152,27.5800026164232,27.6770619121749,27.7740624149263,
27.8710350587886,27.9718597646113,28.0689211634457,28.1660361050485,28.2632831532614,
28.2743338820794),.UNSPECIFIED.);
#595=B_SPLINE_CURVE_WITH_KNOTS('',3,(#58365,#58366,#58367,#58368,#58369,
#58370),.UNSPECIFIED.,.F.,.F.,(4,1,1,4),(15.707963267949,16.3962997518162,
17.3951362017781,17.9335273553052),.UNSPECIFIED.);
#596=B_SPLINE_CURVE_WITH_KNOTS('',3,(#58372,#58373,#58374,#58375,#58376),
 .UNSPECIFIED.,.F.,.F.,(4,1,4),(14.3986268518925,15.3974633018543,15.707963267949),
 .UNSPECIFIED.);
#597=B_SPLINE_CURVE_WITH_KNOTS('',3,(#58380,#58381,#58382,#58383,#58384,
#58385,#58386,#58387,#58388,#58389,#58390,#58391,#58392,#58393,#58394,#58395,
#58396,#58397,#58398,#58399,#58400,#58401,#58402,#58403,#58404,#58405,#58406,
#58407,#58408,#58409,#58410,#58411,#58412,#58413,#58414,#58415,#58416,#58417,
#58418,#58419,#58420,#58421,#58422,#58423,#58424,#58425,#58426,#58427,#58428,
#58429,#58430,#58431,#58432,#58433,#58434,#58435,#58436,#58437),
 .UNSPECIFIED.,.F.,.F.,(4,3,3,3,3,3,3,3,3,3,3,3,3,3,3,3,3,3,3,4),(13.8757070305517,
13.9742335889647,14.072619844817,14.1714715622663,14.2696802945035,14.3678559192405,
14.4660280130677,14.5653794059038,14.6636894122209,14.7635614983165,14.8634335844121,
14.9606976622509,15.0578044027615,15.1548229002686,15.2517842042296,15.3487192914879,
15.4457083558909,15.5427241566488,15.6398692495935,15.707963267949),
 .UNSPECIFIED.);
#598=B_SPLINE_CURVE_WITH_KNOTS('',3,(#58438,#58439,#58440,#58441,#58442,
#58443,#58444),.UNSPECIFIED.,.F.,.F.,(4,1,1,1,4),(15.707963267949,15.8622700343739,
16.8611064843358,17.8599429342977,17.9342415897067),.UNSPECIFIED.);
#599=B_SPLINE_CURVE_WITH_KNOTS('',3,(#58450,#58451,#58452,#58453,#58454,
#58455,#58456,#58457),.UNSPECIFIED.,.F.,.F.,(4,1,1,1,1,4),(181.295997105629,
181.669120728045,182.667957178007,183.666793627969,184.665630077931,185.353966561798),
 .UNSPECIFIED.);
#600=B_SPLINE_CURVE_WITH_KNOTS('',3,(#58459,#58460,#58461,#58462,#58463),
 .UNSPECIFIED.,.F.,.F.,(4,1,4),(185.353966561798,185.664466527893,186.663302977854),
 .UNSPECIFIED.);
#601=B_SPLINE_CURVE_WITH_KNOTS('',3,(#58467,#58468,#58469,#58470,#58471,
#58472,#58473,#58474,#58475,#58476,#58477,#58478,#58479,#58480,#58481,#58482,
#58483,#58484,#58485,#58486,#58487,#58488,#58489,#58490,#58491,#58492,#58493,
#58494,#58495,#58496,#58497,#58498,#58499,#58500,#58501,#58502,#58503,#58504,
#58505,#58506,#58507,#58508,#58509,#58510,#58511,#58512,#58513,#58514,#58515,
#58516,#58517,#58518,#58519,#58520,#58521,#58522,#58523,#58524),
 .UNSPECIFIED.,.F.,.F.,(4,3,3,3,3,3,3,3,3,3,3,3,3,3,3,3,3,3,3,4),(185.353966561798,
185.451129862355,185.548173545581,185.645152144533,185.742096651447,185.839038013602,
185.93606867674,186.033145889087,186.130383557083,186.198496245335,186.297012011071,
186.39538977669,186.494243904503,186.592449804335,186.690624726039,186.788798244729,
186.888154383345,186.9864710254,187.086346912297,187.186222799194),
 .UNSPECIFIED.);
#602=B_SPLINE_CURVE_WITH_KNOTS('',3,(#58525,#58526,#58527,#58528,#58529,
#58530,#58531,#58532),.UNSPECIFIED.,.F.,.F.,(4,1,1,1,1,4),(181.297167536261,
182.203150445487,183.201986895449,184.200823345411,185.199659795373,185.353966561798),
 .UNSPECIFIED.);
#603=B_SPLINE_CURVE_WITH_KNOTS('',3,(#58538,#58539,#58540,#58541,#58542,
#58543,#58544,#58545,#58546,#58547,#58548,#58549,#58550,#58551,#58552,#58553,
#58554,#58555,#58556,#58557,#58558,#58559,#58560,#58561,#58562,#58563,#58564,
#58565,#58566,#58567,#58568,#58569,#58570,#58571,#58572,#58573,#58574,#58575,
#58576,#58577,#58578,#58579,#58580,#58581,#58582,#58583,#58584,#58585,#58586,
#58587,#58588,#58589,#58590,#58591,#58592,#58593,#58594,#58595,#58596,#58597,
#58598,#58599,#58600,#58601,#58602,#58603,#58604,#58605,#58606,#58607,#58608,
#58609,#58610,#58611,#58612,#58613,#58614,#58615,#58616,#58617,#58618,#58619,
#58620,#58621,#58622,#58623,#58624,#58625,#58626,#58627,#58628,#58629,#58630,
#58631,#58632,#58633,#58634,#58635,#58636,#58637,#58638,#58639,#58640,#58641,
#58642,#58643,#58644,#58645,#58646,#58647,#58648,#58649,#58650,#58651,#58652,
#58653,#58654,#58655,#58656,#58657,#58658,#58659,#58660,#58661),
 .UNSPECIFIED.,.F.,.F.,(4,3,3,3,3,3,3,3,3,3,3,3,3,3,3,3,3,3,3,3,3,3,3,3,
3,3,3,3,3,3,3,3,3,3,3,3,3,3,3,3,3,4),(175.013888639089,175.112152299112,
175.210394785152,175.308645570523,175.40699968229,175.505407740544,175.60398608652,
175.676102028274,175.774697487766,175.873152601892,175.973375836435,176.07165273689,
176.169896668633,176.268137117691,176.369837457827,176.468219297092,176.571578887664,
176.674938478236,176.773539091296,176.87199934651,176.972221294221,177.070503268971,
177.168752239357,177.266997685028,177.36869199582,177.4670786771,177.570426802649,
177.673774928198,177.772377760441,177.870840294725,177.971061680154,178.069346062747,
178.167597483387,178.265845418215,178.367536908201,178.465926148849,178.569268763504,
178.672611378159,178.782250126366,178.891545491967,179.000249383586,179.070781030157),
 .UNSPECIFIED.);
#604=B_SPLINE_CURVE_WITH_KNOTS('',3,(#58662,#58663,#58664,#58665,#58666,
#58667),.UNSPECIFIED.,.F.,.F.,(4,1,1,4),(179.070781254618,179.671447828121,
180.670284278083,181.295997105629),.UNSPECIFIED.);
#605=B_SPLINE_CURVE_WITH_KNOTS('',3,(#58669,#58670,#58671,#58672,#58673,
#58674,#58675),.UNSPECIFIED.,.F.,.F.,(4,1,1,1,4),(179.070781254618,179.206641095602,
180.205477545564,181.204313995525,181.297167536261),.UNSPECIFIED.);
#606=B_SPLINE_CURVE_WITH_KNOTS('',3,(#58676,#58677,#58678,#58679,#58680,
#58681,#58682,#58683),.UNSPECIFIED.,.F.,.F.,(4,1,1,1,1,4),(175.01254480072,
175.211295295754,176.210131745716,177.208968195678,178.20780464564,179.070781254618),
 .UNSPECIFIED.);
#607=B_SPLINE_CURVE_WITH_KNOTS('',3,(#58689,#58690,#58691,#58692,#58693,
#58694,#58695,#58696,#58697,#58698,#58699,#58700,#58701,#58702,#58703,#58704,
#58705,#58706,#58707,#58708,#58709,#58710,#58711,#58712,#58713,#58714,#58715,
#58716,#58717,#58718,#58719,#58720,#58721,#58722,#58723,#58724,#58725,#58726,
#58727,#58728,#58729,#58730,#58731,#58732,#58733,#58734,#58735,#58736,#58737,
#58738,#58739,#58740,#58741,#58742,#58743,#58744,#58745,#58746,#58747,#58748,
#58749,#58750,#58751,#58752,#58753,#58754,#58755,#58756,#58757,#58758,#58759,
#58760,#58761,#58762,#58763,#58764,#58765,#58766,#58767,#58768,#58769,#58770,
#58771,#58772,#58773,#58774,#58775,#58776,#58777,#58778,#58779,#58780,#58781,
#58782,#58783,#58784,#58785,#58786,#58787,#58788,#58789,#58790,#58791,#58792,
#58793,#58794,#58795,#58796,#58797,#58798,#58799,#58800,#58801,#58802,#58803,
#58804,#58805,#58806,#58807,#58808,#58809,#58810,#58811,#58812),
 .UNSPECIFIED.,.F.,.F.,(4,3,3,3,3,3,3,3,3,3,3,3,3,3,3,3,3,3,3,3,3,3,3,3,
3,3,3,3,3,3,3,3,3,3,3,3,3,3,3,3,3,4),(168.730499527606,168.829027770498,
168.927431080463,169.025741388665,169.124002483085,169.222243864512,169.320495006626,
169.418850351426,169.51726095759,169.615840356468,169.683083328503,169.781681404593,
169.880139138462,169.980361718462,170.078641227646,170.176887758415,170.275130793449,
170.376828039703,170.47521240635,170.578566092407,170.681919778464,170.780517924859,
170.878975728637,170.979198291111,171.07747786875,171.175724467288,171.273967569322,
171.375664734098,171.474049165163,171.577402696795,171.680756228426,171.7793544904,
171.877812410935,171.978034944366,172.07631464078,172.174561358581,172.272804580209,
172.374501604754,172.472886155,172.576239416694,172.679592678388,172.787595947439),
 .UNSPECIFIED.);
#608=B_SPLINE_CURVE_WITH_KNOTS('',3,(#58813,#58814,#58815,#58816,#58817,
#58818,#58819,#58820,#58821,#58822,#58823,#58824,#58825,#58826,#58827,#58828,
#58829,#58830,#58831,#58832,#58833,#58834,#58835,#58836,#58837,#58838,#58839,
#58840,#58841,#58842,#58843,#58844,#58845,#58846,#58847,#58848,#58849,#58850,
#58851,#58852,#58853,#58854,#58855,#58856,#58857,#58858,#58859,#58860,#58861,
#58862,#58863,#58864,#58865,#58866,#58867,#58868,#58869,#58870,#58871,#58872,
#58873,#58874,#58875,#58876,#58877,#58878,#58879,#58880,#58881,#58882,#58883,
#58884,#58885),.UNSPECIFIED.,.F.,.F.,(4,3,3,3,3,3,3,3,3,3,3,3,3,3,3,3,3,
3,3,3,3,3,3,3,4),(172.787595947668,172.884841558898,172.98404000508,173.081071837534,
173.178059269357,173.275033213409,173.375882192145,173.472980625916,173.570144969666,
173.667458407301,173.67842912835,173.777027506426,173.875485539767,173.975708044585,
174.073987845019,174.172234663368,174.270477981962,174.372174881049,174.470559518455,
174.573912548384,174.677265578312,174.775844827615,174.874301066636,174.972645512634,
175.013888639089),.UNSPECIFIED.);
#609=B_SPLINE_CURVE_WITH_KNOTS('',3,(#58887,#58888,#58889,#58890,#58891,
#58892),.UNSPECIFIED.,.F.,.F.,(4,1,1,4),(172.787601414895,173.21362239583,
174.212458845792,175.01254480072),.UNSPECIFIED.);
#610=B_SPLINE_CURVE_WITH_KNOTS('',3,(#58893,#58894,#58895,#58896,#58897,
#58898,#58899,#58900,#58901,#58902,#58903,#58904,#58905,#58906,#58907,#58908,
#58909,#58910,#58911,#58912,#58913,#58914,#58915,#58916,#58917,#58918,#58919,
#58920,#58921,#58922,#58923,#58924,#58925,#58926,#58927,#58928,#58929,#58930,
#58931,#58932,#58933,#58934,#58935,#58936,#58937,#58938,#58939,#58940,#58941,
#58942,#58943,#58944,#58945,#58946,#58947,#58948,#58949,#58950,#58951,#58952,
#58953,#58954,#58955,#58956,#58957,#58958,#58959,#58960,#58961,#58962,#58963,
#58964,#58965,#58966,#58967,#58968,#58969,#58970,#58971,#58972,#58973,#58974,
#58975,#58976,#58977,#58978,#58979,#58980,#58981,#58982,#58983,#58984,#58985,
#58986,#58987,#58988,#58989,#58990,#58991,#58992,#58993,#58994,#58995,#58996,
#58997,#58998,#58999,#59000,#59001,#59002,#59003,#59004,#59005,#59006,#59007,
#59008,#59009,#59010,#59011,#59012,#59013,#59014,#59015,#59016),
 .UNSPECIFIED.,.F.,.F.,(4,3,3,3,3,3,3,3,3,3,3,3,3,3,3,3,3,3,3,3,3,3,3,3,
3,3,3,3,3,3,3,3,3,3,3,3,3,3,3,3,3,4),(168.730215079385,168.828460546878,
168.926805255148,169.02519788847,169.123767925033,169.218276595983,169.316874714587,
169.41533249097,169.515555060342,169.613834611735,169.71208118451,169.810324261293,
169.912021457456,170.010405864791,170.113759455368,170.217113045945,170.31571117192,
170.41416895561,170.514391523147,170.61267108164,170.710917661422,170.809160745111,
170.91085793281,171.009242346733,171.11259592132,171.215949495907,171.314547642641,
171.413005447249,171.513228009576,171.611507589225,171.709754190205,171.807997295108,
171.909694457798,172.008078892752,172.11143241931,172.214785945869,172.315617765141,
172.416285943305,172.516781875028,172.617176498107,172.717484579422,172.787595947439),
 .UNSPECIFIED.);
#611=B_SPLINE_CURVE_WITH_KNOTS('',3,(#59022,#59023,#59024,#59025,#59026,
#59027,#59028,#59029),.UNSPECIFIED.,.F.,.F.,(4,1,1,1,1,4),(162.446146712717,
162.691228178769,163.690064628731,164.688901078693,165.687737528655,166.504405683028),
 .UNSPECIFIED.);
#612=B_SPLINE_CURVE_WITH_KNOTS('',3,(#59030,#59031,#59032,#59033,#59034,
#59035,#59036,#59037,#59038,#59039,#59040,#59041,#59042,#59043,#59044,#59045,
#59046,#59047,#59048,#59049,#59050,#59051,#59052,#59053,#59054,#59055,#59056,
#59057,#59058,#59059,#59060,#59061,#59062,#59063,#59064,#59065,#59066,#59067,
#59068,#59069,#59070,#59071,#59072,#59073,#59074,#59075,#59076,#59077,#59078,
#59079,#59080,#59081,#59082,#59083,#59084,#59085,#59086,#59087,#59088,#59089,
#59090,#59091,#59092,#59093,#59094,#59095,#59096,#59097,#59098,#59099),
 .UNSPECIFIED.,.F.,.F.,(4,3,3,3,3,3,3,3,3,3,3,3,3,3,3,3,3,3,3,3,3,3,3,4),
(166.504410640259,166.65291077017,166.686573978617,166.785172097224,166.883629873609,
166.983852442981,167.082131994377,167.180378567154,167.278621643939,167.380318840099,
167.478703247436,167.582056838008,167.685410428579,167.784008554555,167.882466338245,
167.982688905782,168.080968464275,168.179215044057,168.277458127747,168.379155315446,
168.477539729369,168.580893303955,168.684246878541,168.730499527606),
 .UNSPECIFIED.);
#613=B_SPLINE_CURVE_WITH_KNOTS('',3,(#59101,#59102,#59103,#59104,#59105,
#59106,#59107,#59108,#59109,#59110,#59111,#59112,#59113,#59114,#59115,#59116,
#59117,#59118,#59119,#59120,#59121,#59122,#59123,#59124,#59125,#59126,#59127,
#59128,#59129,#59130,#59131,#59132,#59133,#59134,#59135,#59136,#59137,#59138,
#59139,#59140,#59141,#59142,#59143,#59144,#59145,#59146,#59147,#59148,#59149,
#59150,#59151,#59152,#59153,#59154,#59155,#59156,#59157,#59158,#59159,#59160,
#59161,#59162,#59163,#59164,#59165,#59166,#59167,#59168,#59169,#59170,#59171,
#59172,#59173),.UNSPECIFIED.,.F.,.F.,(4,3,3,3,3,3,3,3,3,3,3,3,3,3,3,3,3,
3,3,3,3,3,3,3,4),(166.504410640259,166.601913126298,166.699371433805,166.796815990355,
166.894277201717,166.99184617322,167.089478292227,167.187269535427,167.220603696059,
167.319201820913,167.417659603532,167.517882171343,167.616161728894,167.714408307783,
167.81265139063,167.914348579478,168.012732992691,168.116086569356,168.219440146021,
168.31803679311,168.421081364679,168.519419916002,168.61769169675,168.715928369161,
168.730215079385),.UNSPECIFIED.);
#614=B_SPLINE_CURVE_WITH_KNOTS('',3,(#59174,#59175,#59176,#59177,#59178,
#59179,#59180,#59181,#59182,#59183,#59184,#59185,#59186,#59187,#59188,#59189,
#59190,#59191,#59192,#59193,#59194,#59195,#59196,#59197,#59198,#59199,#59200,
#59201,#59202,#59203,#59204,#59205,#59206,#59207,#59208,#59209,#59210,#59211,
#59212,#59213,#59214,#59215,#59216,#59217,#59218,#59219,#59220,#59221,#59222,
#59223,#59224,#59225,#59226,#59227,#59228,#59229,#59230,#59231,#59232,#59233,
#59234,#59235,#59236,#59237,#59238,#59239,#59240,#59241,#59242,#59243,#59244,
#59245,#59246,#59247,#59248,#59249,#59250,#59251,#59252,#59253,#59254,#59255,
#59256,#59257,#59258,#59259,#59260,#59261,#59262,#59263,#59264,#59265,#59266,
#59267,#59268,#59269,#59270,#59271,#59272,#59273,#59274,#59275,#59276,#59277,
#59278,#59279,#59280,#59281,#59282,#59283,#59284,#59285,#59286,#59287,#59288,
#59289,#59290,#59291,#59292,#59293,#59294,#59295,#59296,#59297),
 .UNSPECIFIED.,.F.,.F.,(4,3,3,3,3,3,3,3,3,3,3,3,3,3,3,3,3,3,3,3,3,3,3,3,
3,3,3,3,3,3,3,3,3,3,3,3,3,3,3,3,3,4),(162.447662215674,162.545987512034,
162.644257006383,162.742500209215,162.84074659799,162.939093212585,163.037489181463,
163.136060839186,163.225257896212,163.323856021116,163.422313803793,163.52253637159,
163.62081592922,163.719062508196,163.817305591137,163.919002779896,164.017387193222,
164.120740769698,164.224094346174,164.322692471117,164.421150253833,164.52137282162,
164.619652379284,164.717898958293,164.816142041266,164.917839229983,165.016223643335,
165.119577219736,165.222930796136,165.321528921637,165.419986704913,165.520209272561,
165.618488830789,165.71673541036,165.814978493895,165.916675681946,166.015060095852,
166.118413670974,166.221767246097,166.344599874398,166.465474953135,166.504410639987),
 .UNSPECIFIED.);
#615=B_SPLINE_CURVE_WITH_KNOTS('',3,(#59303,#59304,#59305,#59306,#59307,
#59308,#59309,#59310,#59311,#59312,#59313,#59314,#59315,#59316,#59317,#59318,
#59319,#59320,#59321,#59322,#59323,#59324,#59325,#59326,#59327,#59328,#59329,
#59330,#59331,#59332,#59333,#59334,#59335,#59336,#59337,#59338,#59339,#59340,
#59341,#59342,#59343,#59344,#59345,#59346,#59347,#59348,#59349,#59350,#59351,
#59352,#59353,#59354,#59355,#59356,#59357,#59358,#59359,#59360,#59361,#59362,
#59363,#59364,#59365,#59366,#59367,#59368,#59369,#59370,#59371,#59372,#59373,
#59374,#59375,#59376,#59377,#59378,#59379,#59380,#59381,#59382,#59383,#59384,
#59385,#59386,#59387,#59388,#59389,#59390,#59391,#59392,#59393,#59394,#59395,
#59396,#59397,#59398,#59399,#59400,#59401,#59402,#59403,#59404,#59405,#59406,
#59407,#59408,#59409,#59410,#59411,#59412,#59413,#59414,#59415,#59416,#59417,
#59418,#59419,#59420,#59421,#59422,#59423,#59424,#59425,#59426,#59427,#59428,
#59429),.UNSPECIFIED.,.F.,.F.,(4,3,3,3,3,3,3,3,3,3,3,3,3,3,3,3,3,3,3,3,
3,3,3,3,3,3,3,3,3,3,3,3,3,3,3,3,3,3,3,3,3,3,4),(156.163987574067,156.262228618507,
156.360486880375,156.458853673816,156.557282430391,156.655872527635,156.698209478998,
156.796807604012,156.895265386799,156.995487954569,157.093767512308,157.192014091391,
157.29025717444,157.39195436307,157.490338776499,157.593692352729,157.69704592896,
157.795644053952,157.894101836717,157.994324404492,158.092603962209,158.190850541271,
158.289093624298,158.390790812954,158.489175226362,158.592528802642,158.695882378922,
158.794480503912,158.892938286674,158.993160854451,159.091440412165,159.189686991223,
159.287930074248,159.389627262907,159.488011676311,159.591365252598,159.694718828884,
159.797216560019,159.903218753284,160.005303397592,160.107256278838,160.209067828957,
160.22122533308),.UNSPECIFIED.);
#616=B_SPLINE_CURVE_WITH_KNOTS('',3,(#59430,#59431,#59432,#59433,#59434,
#59435),.UNSPECIFIED.,.F.,.F.,(4,1,1,4),(160.221227414851,160.693555278846,
161.692391728808,162.446146712717),.UNSPECIFIED.);
#617=B_SPLINE_CURVE_WITH_KNOTS('',3,(#59437,#59438,#59439,#59440,#59441,
#59442,#59443,#59444,#59445,#59446,#59447,#59448,#59449,#59450,#59451,#59452,
#59453,#59454,#59455,#59456,#59457,#59458,#59459,#59460,#59461,#59462,#59463,
#59464,#59465,#59466,#59467,#59468,#59469,#59470,#59471,#59472,#59473,#59474,
#59475,#59476,#59477,#59478,#59479,#59480,#59481,#59482,#59483,#59484,#59485,
#59486,#59487,#59488,#59489,#59490,#59491,#59492,#59493,#59494,#59495,#59496,
#59497,#59498,#59499,#59500,#59501,#59502,#59503,#59504,#59505,#59506,#59507,
#59508,#59509),.UNSPECIFIED.,.F.,.F.,(4,3,3,3,3,3,3,3,3,3,3,3,3,3,3,3,3,
3,3,3,3,3,3,3,4),(160.22122533308,160.228748546326,160.327346671318,160.425804454083,
160.526027021859,160.624306579575,160.722553158637,160.820796241664,160.92249343032,
161.020877843728,161.124231420008,161.227584996288,161.326183121278,161.424640904041,
161.524863471817,161.623143029531,161.72138960859,161.819632691614,161.921329880273,
162.019714293677,162.123067869964,162.22642144625,162.325027405988,162.423481500074,
162.447662215674),.UNSPECIFIED.);
#618=B_SPLINE_CURVE_WITH_KNOTS('',3,(#59510,#59511,#59512,#59513,#59514,
#59515,#59516,#59517,#59518,#59519,#59520,#59521,#59522,#59523,#59524,#59525,
#59526,#59527,#59528,#59529,#59530,#59531,#59532,#59533,#59534,#59535,#59536,
#59537,#59538,#59539,#59540,#59541,#59542,#59543,#59544,#59545,#59546,#59547,
#59548,#59549,#59550,#59551,#59552,#59553,#59554,#59555,#59556,#59557,#59558,
#59559,#59560,#59561,#59562,#59563,#59564,#59565,#59566,#59567,#59568,#59569,
#59570,#59571,#59572,#59573,#59574,#59575,#59576,#59577,#59578,#59579,#59580,
#59581,#59582,#59583,#59584,#59585,#59586,#59587,#59588,#59589,#59590,#59591,
#59592,#59593,#59594,#59595,#59596,#59597,#59598,#59599,#59600,#59601,#59602,
#59603,#59604,#59605,#59606,#59607,#59608,#59609,#59610,#59611,#59612,#59613,
#59614,#59615,#59616,#59617,#59618,#59619,#59620,#59621,#59622,#59623,#59624,
#59625,#59626,#59627,#59628,#59629,#59630,#59631,#59632,#59633),
 .UNSPECIFIED.,.F.,.F.,(4,3,3,3,3,3,3,3,3,3,3,3,3,3,3,3,3,3,3,3,3,3,3,3,
3,3,3,3,3,3,3,3,3,3,3,3,3,3,3,3,3,4),(156.163531910326,156.233402746479,
156.332000871484,156.430458654262,156.530681222035,156.628960779764,156.727207358839,
156.825450441879,156.927147630519,157.02553204394,157.12888562019,157.232239196441,
157.330837321443,157.429295104219,157.529517671992,157.627797229718,157.72604380879,
157.824286891828,157.925984080471,158.024368493889,158.127722070145,158.231075646402,
158.329673771403,158.428131554177,158.52835412195,158.626633679676,158.724880258747,
158.823123341782,158.924820530428,159.023204943844,159.126558520104,159.229912096364,
159.328378576654,159.426704810661,159.526019875932,159.624169149678,159.722285836342,
159.820399593048,159.920606027993,160.018861091251,160.120043212039,160.221225332828),
 .UNSPECIFIED.);
#619=B_SPLINE_CURVE_WITH_KNOTS('',3,(#59639,#59640,#59641,#59642,#59643,
#59644,#59645,#59646),.UNSPECIFIED.,.F.,.F.,(4,1,1,1,1,4),(149.881541683267,
150.705190779227,151.704027229189,152.702863679151,153.701700129113,153.938039726484),
 .UNSPECIFIED.);
#620=B_SPLINE_CURVE_WITH_KNOTS('',3,(#59647,#59648,#59649,#59650,#59651,
#59652,#59653,#59654,#59655,#59656,#59657,#59658,#59659,#59660,#59661,#59662,
#59663,#59664,#59665,#59666,#59667,#59668,#59669,#59670,#59671,#59672,#59673,
#59674,#59675,#59676,#59677,#59678,#59679,#59680,#59681,#59682,#59683,#59684,
#59685,#59686,#59687,#59688,#59689,#59690,#59691,#59692,#59693,#59694,#59695,
#59696,#59697,#59698,#59699,#59700,#59701,#59702,#59703,#59704,#59705,#59706,
#59707,#59708,#59709,#59710,#59711,#59712,#59713,#59714,#59715,#59716),
 .UNSPECIFIED.,.F.,.F.,(4,3,3,3,3,3,3,3,3,3,3,3,3,3,3,3,3,3,3,3,3,3,3,4),
(153.9380400259,154.035163898234,154.132222574362,154.229246955324,154.326267897773,
154.423381488606,154.520541056366,154.617870832504,154.700536579074,154.799134704076,
154.897592486852,154.997815054625,155.096094612352,155.194341191424,155.292584274461,
155.394281463105,155.492665876522,155.596019452779,155.699373029036,155.797975862223,
155.896415143035,155.994759399106,156.093038592393,156.163987574067),
 .UNSPECIFIED.);
#621=B_SPLINE_CURVE_WITH_KNOTS('',3,(#59718,#59719,#59720,#59721,#59722,
#59723,#59724,#59725,#59726,#59727,#59728,#59729,#59730,#59731,#59732,#59733,
#59734,#59735,#59736,#59737,#59738,#59739,#59740,#59741,#59742,#59743,#59744,
#59745,#59746,#59747,#59748,#59749,#59750,#59751,#59752,#59753,#59754,#59755,
#59756,#59757,#59758,#59759,#59760,#59761,#59762,#59763,#59764,#59765,#59766,
#59767,#59768,#59769,#59770,#59771,#59772,#59773,#59774,#59775,#59776,#59777,
#59778,#59779,#59780,#59781,#59782,#59783,#59784,#59785,#59786,#59787),
 .UNSPECIFIED.,.F.,.F.,(4,3,3,3,3,3,3,3,3,3,3,3,3,3,3,3,3,3,3,3,3,3,3,4),
(153.938040202782,154.056659980249,154.176963651006,154.235729846555,154.334327971559,
154.432785754335,154.533008322108,154.631287879836,154.729534458909,154.827777541948,
154.92947473059,155.027859144009,155.131212720263,155.234566296517,155.333169148011,
155.431630381049,155.5299726517,155.628250049483,155.726492098718,155.824728281928,
155.923038846784,156.021391522265,156.119876942697,156.163531910326),
 .UNSPECIFIED.);
#622=B_SPLINE_CURVE_WITH_KNOTS('',3,(#59788,#59789,#59790,#59791,#59792,
#59793,#59794,#59795),.UNSPECIFIED.,.F.,.F.,(4,1,1,1,1,4),(149.880018474884,
150.240384046707,151.239220496669,152.238056946631,153.236893396593,153.9380400259),
 .UNSPECIFIED.);
#623=B_SPLINE_CURVE_WITH_KNOTS('',3,(#59801,#59802,#59803,#59804,#59805,
#59806,#59807,#59808,#59809,#59810,#59811,#59812,#59813,#59814,#59815,#59816,
#59817,#59818,#59819,#59820,#59821,#59822,#59823,#59824,#59825,#59826,#59827,
#59828,#59829,#59830,#59831,#59832,#59833,#59834,#59835,#59836,#59837,#59838,
#59839,#59840,#59841,#59842,#59843,#59844,#59845,#59846,#59847,#59848,#59849,
#59850,#59851,#59852,#59853,#59854,#59855,#59856,#59857,#59858,#59859,#59860,
#59861,#59862,#59863,#59864,#59865,#59866,#59867,#59868,#59869,#59870,#59871,
#59872,#59873,#59874,#59875,#59876,#59877,#59878,#59879,#59880,#59881,#59882,
#59883,#59884,#59885,#59886,#59887,#59888,#59889,#59890,#59891,#59892,#59893,
#59894,#59895,#59896,#59897,#59898,#59899,#59900,#59901,#59902,#59903,#59904,
#59905,#59906,#59907,#59908,#59909,#59910,#59911,#59912,#59913,#59914,#59915,
#59916,#59917,#59918,#59919,#59920,#59921,#59922,#59923,#59924,#59925,#59926,
#59927),.UNSPECIFIED.,.F.,.F.,(4,3,3,3,3,3,3,3,3,3,3,3,3,3,3,3,3,3,3,3,
3,3,3,3,3,3,3,3,3,3,3,3,3,3,3,3,3,3,3,3,3,3,4),(143.59701849018,143.69562123255,
143.713335629494,143.811933754498,143.910391537275,144.010614105047,144.108893662775,
144.207140241849,144.305383324887,144.40708051353,144.505464926948,144.608818503202,
144.712172079456,144.81077020446,144.909227987236,145.009450555009,145.107730112737,
145.205976691811,145.304219774849,145.405916963491,145.50430137691,145.607654953164,
145.711008529418,145.809606654422,145.908064437198,146.008287004971,146.106566562699,
146.204813141772,146.303056224811,146.404753413453,146.503137826872,146.606491403125,
146.709844979379,146.807643480436,146.905302408374,147.002849316603,147.100335701354,
147.197792033696,147.295248746519,147.3927980835,147.490396206244,147.588155506493,
147.65485471872),.UNSPECIFIED.);
#624=B_SPLINE_CURVE_WITH_KNOTS('',3,(#59928,#59929,#59930,#59931,#59932,
#59933,#59934),.UNSPECIFIED.,.F.,.F.,(4,1,1,1,4),(147.65485471872,147.708681429341,
148.707517879303,149.706354329265,149.881541683267),.UNSPECIFIED.);
#625=B_SPLINE_CURVE_WITH_KNOTS('',3,(#59936,#59937,#59938,#59939,#59940,
#59941),.UNSPECIFIED.,.F.,.F.,(4,1,1,4),(147.65485471872,148.242711146784,
149.241547596746,149.880018474884),.UNSPECIFIED.);
#626=B_SPLINE_CURVE_WITH_KNOTS('',3,(#59942,#59943,#59944,#59945,#59946,
#59947,#59948,#59949,#59950,#59951,#59952,#59953,#59954,#59955,#59956,#59957,
#59958,#59959,#59960,#59961,#59962,#59963,#59964,#59965,#59966,#59967,#59968,
#59969,#59970,#59971,#59972,#59973,#59974,#59975,#59976,#59977,#59978,#59979,
#59980,#59981,#59982,#59983,#59984,#59985,#59986,#59987,#59988,#59989,#59990,
#59991,#59992,#59993,#59994,#59995,#59996,#59997,#59998,#59999,#60000,#60001,
#60002,#60003,#60004,#60005,#60006,#60007,#60008,#60009,#60010,#60011,#60012,
#60013,#60014,#60015,#60016,#60017,#60018,#60019,#60020,#60021,#60022,#60023,
#60024,#60025,#60026,#60027,#60028,#60029,#60030,#60031,#60032,#60033,#60034,
#60035,#60036,#60037,#60038,#60039,#60040,#60041,#60042,#60043,#60044,#60045,
#60046,#60047,#60048,#60049,#60050,#60051,#60052,#60053,#60054,#60055,#60056,
#60057,#60058,#60059,#60060,#60061,#60062,#60063,#60064,#60065),
 .UNSPECIFIED.,.F.,.F.,(4,3,3,3,3,3,3,3,3,3,3,3,3,3,3,3,3,3,3,3,3,3,3,3,
3,3,3,3,3,3,3,3,3,3,3,3,3,3,3,3,3,4),(143.597933903879,143.6961922985,143.794433353168,
143.892686540564,143.991045328786,144.089461510033,144.188044071276,144.247365346936,
144.34596347194,144.444421254717,144.544643822489,144.642923380217,144.741169959291,
144.839413042329,144.941110230972,145.03949464439,145.142848220644,145.246201796898,
145.344799921902,145.443257704678,145.543480272451,145.641759830179,145.740006409253,
145.838249492291,145.939946680933,146.038331094352,146.141684670606,146.24503824686,
146.343636371864,146.44209415464,146.542316722413,146.640596280141,146.738842859215,
146.837085942253,146.938783130895,147.037167544314,147.140521120568,147.243874696822,
147.352569174392,147.460952550046,147.568802109382,147.654854305383),
 .UNSPECIFIED.);
#627=B_SPLINE_CURVE_WITH_KNOTS('',3,(#60071,#60072,#60073,#60074,#60075,
#60076,#60077,#60078,#60079,#60080,#60081,#60082,#60083,#60084,#60085,#60086,
#60087,#60088,#60089,#60090,#60091,#60092,#60093,#60094,#60095,#60096,#60097,
#60098,#60099,#60100,#60101,#60102,#60103,#60104,#60105,#60106,#60107,#60108,
#60109,#60110,#60111,#60112,#60113,#60114,#60115,#60116,#60117,#60118,#60119,
#60120,#60121,#60122,#60123,#60124,#60125,#60126,#60127,#60128,#60129,#60130,
#60131,#60132,#60133,#60134,#60135,#60136,#60137,#60138,#60139,#60140,#60141,
#60142,#60143,#60144,#60145,#60146,#60147,#60148,#60149,#60150,#60151,#60152,
#60153,#60154,#60155,#60156,#60157,#60158,#60159,#60160,#60161,#60162,#60163,
#60164,#60165,#60166,#60167,#60168,#60169,#60170,#60171,#60172,#60173,#60174,
#60175,#60176,#60177,#60178,#60179,#60180,#60181,#60182,#60183,#60184,#60185,
#60186,#60187,#60188,#60189,#60190,#60191,#60192,#60193,#60194),
 .UNSPECIFIED.,.F.,.F.,(4,3,3,3,3,3,3,3,3,3,3,3,3,3,3,3,3,3,3,3,3,3,3,3,
3,3,3,3,3,3,3,3,3,3,3,3,3,3,3,3,3,4),(137.314044075445,137.415612289014,
137.513996928846,137.617156929285,137.720316929723,137.818915054727,137.917372837503,
138.017595405276,138.115874963004,138.214121542077,138.312364625116,138.414061813758,
138.512446227177,138.61579980343,138.719153379684,138.817751504687,138.916209287464,
139.016431855237,139.114711412965,139.212957992038,139.311201075077,139.412898263719,
139.511282677138,139.614636253392,139.717989829646,139.81658795465,139.915045737426,
140.015268305199,140.113547862927,140.211794442001,140.310037525039,140.411734713681,
140.5101191271,140.613472703354,140.716826279608,140.815569227393,140.914173010821,
141.012667061739,141.111081830931,141.209449097701,141.307822396311,141.371669411541),
 .UNSPECIFIED.);
#628=B_SPLINE_CURVE_WITH_KNOTS('',3,(#60195,#60196,#60197,#60198,#60199,
#60200,#60201,#60202,#60203,#60204,#60205,#60206,#60207,#60208,#60209,#60210,
#60211,#60212,#60213,#60214,#60215,#60216,#60217,#60218,#60219,#60220,#60221,
#60222,#60223,#60224,#60225,#60226,#60227,#60228,#60229,#60230,#60231,#60232,
#60233,#60234,#60235,#60236,#60237,#60238,#60239,#60240,#60241,#60242,#60243,
#60244,#60245,#60246,#60247,#60248,#60249,#60250,#60251,#60252,#60253,#60254,
#60255,#60256,#60257,#60258,#60259,#60260,#60261),.UNSPECIFIED.,.F.,.F.,
(4,3,3,3,3,3,3,3,3,3,3,3,3,3,3,3,3,3,3,3,3,3,4),(141.371669411768,141.485016004535,
141.600339367052,141.71566272957,141.814260854574,141.912718637351,142.012941205123,
142.111220762851,142.209467341925,142.307710424963,142.409407613606,142.507792027024,
142.611145603278,142.714499179532,142.813105314796,142.911543009966,143.009885026329,
143.108160960054,143.206400336867,143.304679404122,143.402973649647,143.501391759129,
143.59701849018),.UNSPECIFIED.);
#629=B_SPLINE_CURVE_WITH_KNOTS('',3,(#60263,#60264,#60265,#60266,#60267,
#60268,#60269,#60270,#60271,#60272,#60273,#60274,#60275,#60276,#60277,#60278,
#60279,#60280,#60281,#60282,#60283,#60284,#60285,#60286,#60287,#60288,#60289,
#60290,#60291,#60292,#60293,#60294,#60295,#60296,#60297,#60298,#60299,#60300,
#60301,#60302,#60303,#60304,#60305,#60306,#60307,#60308,#60309,#60310,#60311,
#60312,#60313,#60314,#60315,#60316,#60317,#60318,#60319,#60320,#60321,#60322,
#60323,#60324,#60325,#60326,#60327,#60328,#60329,#60330,#60331,#60332),
 .UNSPECIFIED.,.F.,.F.,(4,3,3,3,3,3,3,3,3,3,3,3,3,3,3,3,3,3,3,3,3,3,3,4),
(141.371669411541,141.46883125416,141.566438903267,141.66339620349,141.760311911022,
141.857216996242,141.955335858935,142.052368429038,142.151030438025,142.249692447012,
142.348290572016,142.446748354793,142.546970922565,142.645250480293,142.743497059367,
142.841740142405,142.943437331047,143.041821744466,143.14517532072,143.248528896974,
143.347104955703,143.44555813638,143.543900701717,143.597933903879),
 .UNSPECIFIED.);
#630=B_SPLINE_CURVE_WITH_KNOTS('',3,(#60333,#60334,#60335,#60336,#60337,
#60338,#60339,#60340),.UNSPECIFIED.,.F.,.F.,(4,1,1,1,1,4),(137.314688056577,
138.254346647165,139.253183097127,140.252019547089,141.250855997051,141.371669411541),
 .UNSPECIFIED.);
#631=B_SPLINE_CURVE_WITH_KNOTS('',3,(#60346,#60347,#60348,#60349,#60350,
#60351,#60352,#60353,#60354,#60355,#60356,#60357,#60358,#60359,#60360,#60361,
#60362,#60363,#60364,#60365,#60366,#60367,#60368,#60369,#60370,#60371,#60372,
#60373,#60374,#60375,#60376,#60377,#60378,#60379,#60380,#60381,#60382,#60383,
#60384,#60385,#60386,#60387,#60388,#60389,#60390,#60391,#60392,#60393,#60394,
#60395,#60396,#60397,#60398,#60399,#60400,#60401,#60402,#60403,#60404,#60405,
#60406,#60407,#60408,#60409,#60410,#60411,#60412,#60413,#60414,#60415,#60416,
#60417,#60418,#60419,#60420,#60421,#60422,#60423,#60424,#60425,#60426,#60427,
#60428,#60429,#60430,#60431,#60432,#60433,#60434,#60435,#60436,#60437,#60438,
#60439,#60440,#60441,#60442,#60443,#60444,#60445,#60446,#60447,#60448,#60449,
#60450,#60451,#60452,#60453,#60454,#60455,#60456,#60457,#60458,#60459,#60460,
#60461,#60462,#60463,#60464,#60465,#60466,#60467,#60468,#60469),
 .UNSPECIFIED.,.F.,.F.,(4,3,3,3,3,3,3,3,3,3,3,3,3,3,3,3,3,3,3,3,3,3,3,3,
3,3,3,3,3,3,3,3,3,3,3,3,3,3,3,3,3,4),(131.031654953742,131.129931693063,
131.228177228462,131.326421041054,131.426640338278,131.525027370655,131.626162800303,
131.727298229951,131.825896354955,131.924354137731,132.024576705504,132.122856263232,
132.221102842306,132.319345925344,132.421043113987,132.519427527405,132.622781103659,
132.726134679913,132.824732804917,132.923190587694,133.023413155466,133.121692713194,
133.219939292268,133.318182375306,133.419879563948,133.518263977367,133.621617553621,
133.724971129875,133.823569254879,133.922027037655,134.022249605428,134.120529163156,
134.218775742229,134.317018825268,134.41871601391,134.517100427329,134.620454003583,
134.723807579837,134.836338520701,134.948409000642,135.059693750752,135.088484104126),
 .UNSPECIFIED.);
#632=B_SPLINE_CURVE_WITH_KNOTS('',3,(#60470,#60471,#60472,#60473,#60474,
#60475,#60476,#60477,#60478,#60479,#60480,#60481,#60482,#60483,#60484,#60485,
#60486,#60487,#60488,#60489,#60490,#60491,#60492,#60493,#60494,#60495,#60496,
#60497,#60498,#60499,#60500,#60501,#60502,#60503,#60504,#60505,#60506,#60507,
#60508,#60509,#60510,#60511,#60512,#60513,#60514,#60515,#60516,#60517,#60518,
#60519,#60520,#60521,#60522,#60523,#60524,#60525,#60526,#60527,#60528,#60529,
#60530,#60531,#60532,#60533,#60534,#60535,#60536,#60537,#60538,#60539),
 .UNSPECIFIED.,.F.,.F.,(4,3,3,3,3,3,3,3,3,3,3,3,3,3,3,3,3,3,3,3,3,3,3,4),
(135.088484104361,135.187254556185,135.286029876603,135.384838499173,135.483776463585,
135.582788468007,135.681976179005,135.722644029799,135.821242154803,135.91969993758,
136.019922505352,136.11820206308,136.216448642154,136.314691725192,136.416388913834,
136.514773327253,136.618126903507,136.721480479761,136.820067256332,136.918521077989,
137.017401827353,137.115677667237,137.214860871341,137.314044075445),
 .UNSPECIFIED.);
#633=B_SPLINE_CURVE_WITH_KNOTS('',3,(#60541,#60542,#60543,#60544,#60545,
#60546,#60547),.UNSPECIFIED.,.F.,.F.,(4,1,1,1,4),(135.088484104361,135.257837297279,
136.256673747241,137.255510197203,137.314688056577),.UNSPECIFIED.);
#634=B_SPLINE_CURVE_WITH_KNOTS('',3,(#60548,#60549,#60550,#60551,#60552,
#60553,#60554,#60555,#60556,#60557,#60558,#60559,#60560,#60561,#60562,#60563,
#60564,#60565,#60566,#60567,#60568,#60569,#60570,#60571,#60572,#60573,#60574,
#60575,#60576,#60577,#60578,#60579,#60580,#60581,#60582,#60583,#60584,#60585,
#60586,#60587,#60588,#60589,#60590,#60591,#60592,#60593,#60594,#60595,#60596,
#60597,#60598,#60599,#60600,#60601,#60602,#60603,#60604,#60605,#60606,#60607,
#60608,#60609,#60610,#60611,#60612,#60613,#60614,#60615,#60616,#60617,#60618,
#60619,#60620,#60621,#60622,#60623,#60624,#60625,#60626,#60627,#60628,#60629,
#60630,#60631,#60632,#60633,#60634,#60635,#60636,#60637,#60638,#60639,#60640,
#60641,#60642,#60643,#60644,#60645,#60646,#60647,#60648,#60649,#60650,#60651,
#60652,#60653,#60654,#60655,#60656,#60657,#60658,#60659,#60660,#60661,#60662,
#60663,#60664,#60665,#60666,#60667,#60668,#60669,#60670,#60671,#60672,#60673,
#60674),.UNSPECIFIED.,.F.,.F.,(4,3,3,3,3,3,3,3,3,3,3,3,3,3,3,3,3,3,3,3,
3,3,3,3,3,3,3,3,3,3,3,3,3,3,3,3,3,3,3,3,3,3,4),(131.03054492507,131.128979421002,
131.227573113898,131.262491497432,131.361089622436,131.459547405213,131.559769972985,
131.658049530713,131.756296109787,131.854539192826,131.956236381468,132.054620794887,
132.15797437114,132.261327947394,132.359926072398,132.458383855174,132.558606422947,
132.656885980675,132.755132559748,132.853375642787,132.955072831429,133.053457244848,
133.156810821102,133.260164397356,133.35876252236,133.457220305136,133.557442872909,
133.655722430637,133.75396900971,133.852212092749,133.953909281391,134.05229369481,
134.155647271063,134.259000847317,134.356128675186,134.453094160804,134.549968416923,
134.646782617699,134.743567858738,134.84039997176,134.937256811786,135.034231214225,
135.088484104361),.UNSPECIFIED.);
#635=B_SPLINE_CURVE_WITH_KNOTS('',3,(#60680,#60681,#60682,#60683,#60684,
#60685,#60686,#60687),.UNSPECIFIED.,.F.,.F.,(4,1,1,1,1,4),(124.748033464244,
125.73427953018,126.733115980142,127.731952430104,128.730788880066,128.805298797182),
 .UNSPECIFIED.);
#636=B_SPLINE_CURVE_WITH_KNOTS('',3,(#60688,#60689,#60690,#60691,#60692,
#60693,#60694,#60695,#60696,#60697,#60698,#60699,#60700,#60701,#60702,#60703,
#60704,#60705,#60706,#60707,#60708,#60709,#60710,#60711,#60712,#60713,#60714,
#60715,#60716,#60717,#60718,#60719,#60720,#60721,#60722,#60723,#60724,#60725,
#60726,#60727,#60728,#60729,#60730,#60731,#60732,#60733,#60734,#60735,#60736,
#60737,#60738,#60739,#60740,#60741,#60742,#60743,#60744,#60745,#60746,#60747,
#60748,#60749,#60750,#60751,#60752,#60753,#60754,#60755,#60756,#60757),
 .UNSPECIFIED.,.F.,.F.,(4,3,3,3,3,3,3,3,3,3,3,3,3,3,3,3,3,3,3,3,3,3,3,4),
(128.805298797182,128.902840431273,129.000250613517,129.097560812666,129.194818343698,
129.292053887498,129.389298094495,129.486642967569,129.584044330746,129.681605924981,
129.729625330028,129.828223455032,129.926681237808,130.026903805581,130.125183363309,
130.223429942382,130.321673025421,130.423370214063,130.521754627482,130.625108203735,
130.728461779989,130.827047027845,130.929350990793,131.031654953742),
 .UNSPECIFIED.);
#637=B_SPLINE_CURVE_WITH_KNOTS('',3,(#60759,#60760,#60761,#60762,#60763,
#60764,#60765,#60766,#60767,#60768,#60769,#60770,#60771,#60772,#60773,#60774,
#60775,#60776,#60777,#60778,#60779,#60780,#60781,#60782,#60783,#60784,#60785,
#60786,#60787,#60788,#60789,#60790,#60791,#60792,#60793,#60794,#60795,#60796,
#60797,#60798,#60799,#60800,#60801,#60802,#60803,#60804,#60805,#60806,#60807,
#60808,#60809,#60810,#60811,#60812,#60813,#60814,#60815,#60816,#60817,#60818,
#60819,#60820,#60821,#60822,#60823,#60824,#60825,#60826,#60827,#60828),
 .UNSPECIFIED.,.F.,.F.,(4,3,3,3,3,3,3,3,3,3,3,3,3,3,3,3,3,3,3,3,3,3,3,4),
(128.805299011168,128.910085619878,129.015255759158,129.12063010964,129.226318351055,
129.264818597508,129.363416722512,129.461874505288,129.562097073061,129.660376630789,
129.758623209863,129.856866292901,129.958563481543,130.056947894962,130.160301471216,
130.26365504747,130.362225486657,130.460667523602,130.559010865893,130.657285118178,
130.755545076205,130.853792579357,130.952108672676,131.03054492507),
 .UNSPECIFIED.);
#638=B_SPLINE_CURVE_WITH_KNOTS('',3,(#60829,#60830,#60831,#60832,#60833,
#60834,#60835,#60836),.UNSPECIFIED.,.F.,.F.,(4,1,1,1,1,4),(124.748072421146,
125.269472797661,126.268309247622,127.267145697584,128.265982147546,128.805298797182),
 .UNSPECIFIED.);
#639=B_SPLINE_CURVE_WITH_KNOTS('',3,(#60842,#60843,#60844,#60845,#60846,
#60847,#60848,#60849,#60850,#60851,#60852,#60853,#60854,#60855,#60856,#60857,
#60858,#60859,#60860,#60861,#60862,#60863,#60864,#60865,#60866,#60867,#60868,
#60869,#60870,#60871,#60872,#60873,#60874,#60875,#60876,#60877,#60878,#60879,
#60880,#60881,#60882,#60883,#60884,#60885,#60886,#60887,#60888,#60889,#60890,
#60891,#60892,#60893,#60894,#60895,#60896,#60897,#60898,#60899,#60900,#60901,
#60902,#60903,#60904,#60905,#60906,#60907,#60908,#60909,#60910,#60911,#60912,
#60913,#60914,#60915,#60916,#60917,#60918,#60919,#60920,#60921,#60922,#60923,
#60924,#60925,#60926,#60927,#60928,#60929,#60930,#60931,#60932,#60933,#60934,
#60935,#60936,#60937,#60938,#60939,#60940,#60941,#60942,#60943,#60944,#60945,
#60946,#60947,#60948,#60949,#60950,#60951,#60952,#60953,#60954,#60955,#60956,
#60957,#60958,#60959,#60960,#60961,#60962,#60963,#60964,#60965),
 .UNSPECIFIED.,.F.,.F.,(4,3,3,3,3,3,3,3,3,3,3,3,3,3,3,3,3,3,3,3,3,3,3,3,
3,3,3,3,3,3,3,3,3,3,3,3,3,3,3,3,3,4),(118.464214588977,118.562615707051,
118.661189977465,118.742424380447,118.841022505451,118.939480288228,119.039702856,
119.137982413728,119.236228992802,119.33447207584,119.436169264482,119.534553677901,
119.637907254155,119.741260830409,119.839858955413,119.93831673819,120.038539305962,
120.136818863691,120.235065442764,120.333308525802,120.435005714445,120.533390127863,
120.636743704117,120.740097280371,120.838695405375,120.937153188151,121.037375755924,
121.135655313652,121.233901892725,121.332144975764,121.433842164406,121.532226577825,
121.635580154079,121.738933730333,121.836831200292,121.933909156543,122.030894120917,
122.127817176648,122.226391254986,122.323316910845,122.422715200424,122.522113490002),
 .UNSPECIFIED.);
#640=B_SPLINE_CURVE_WITH_KNOTS('',3,(#60966,#60967,#60968,#60969,#60970,
#60971,#60972),.UNSPECIFIED.,.F.,.F.,(4,1,1,1,4),(122.522113490002,122.737770180294,
123.736606630256,124.735443080218,124.748033464244),.UNSPECIFIED.);
#641=B_SPLINE_CURVE_WITH_KNOTS('',3,(#60974,#60975,#60976,#60977,#60978,
#60979),.UNSPECIFIED.,.F.,.F.,(4,1,1,4),(122.522113490002,123.271799897737,
124.270636347699,124.748072421146),.UNSPECIFIED.);
#642=B_SPLINE_CURVE_WITH_KNOTS('',3,(#60980,#60981,#60982,#60983,#60984,
#60985,#60986,#60987,#60988,#60989,#60990,#60991,#60992,#60993,#60994,#60995,
#60996,#60997,#60998,#60999,#61000,#61001,#61002,#61003,#61004,#61005,#61006,
#61007,#61008,#61009,#61010,#61011,#61012,#61013,#61014,#61015,#61016,#61017,
#61018,#61019,#61020,#61021,#61022,#61023,#61024,#61025,#61026,#61027,#61028,
#61029,#61030,#61031,#61032,#61033,#61034,#61035,#61036,#61037,#61038,#61039,
#61040,#61041,#61042,#61043,#61044,#61045,#61046,#61047,#61048,#61049,#61050,
#61051,#61052,#61053,#61054,#61055,#61056,#61057,#61058,#61059,#61060,#61061,
#61062,#61063,#61064,#61065,#61066,#61067,#61068,#61069,#61070,#61071,#61072,
#61073,#61074,#61075,#61076,#61077,#61078,#61079,#61080,#61081,#61082,#61083,
#61084,#61085,#61086,#61087,#61088,#61089,#61090,#61091,#61092,#61093,#61094,
#61095,#61096,#61097,#61098,#61099,#61100,#61101,#61102,#61103),
 .UNSPECIFIED.,.F.,.F.,(4,3,3,3,3,3,3,3,3,3,3,3,3,3,3,3,3,3,3,3,3,3,3,3,
3,3,3,3,3,3,3,3,3,3,3,3,3,3,3,3,3,4),(118.465360130437,118.566746876369,
118.665030492148,118.763278683933,118.861520936572,118.959786720207,119.058164549422,
119.156610017844,119.255210823008,119.276454097889,119.375052222893,119.47351000567,
119.573732573442,119.67201213117,119.770258710244,119.868501793282,119.970198981924,
120.068583395343,120.171936971597,120.275290547851,120.373888672855,120.472346455632,
120.572569023404,120.670848581132,120.769095160206,120.867338243244,120.969035431886,
121.067419845305,121.170773421559,121.274126997813,121.372725122817,121.471182905593,
121.571405473366,121.669685031094,121.767931610168,121.866174693206,121.967871881848,
122.066256295267,122.169609871521,122.272963447775,122.400857829824,122.522113389936),
 .UNSPECIFIED.);
#643=B_SPLINE_CURVE_WITH_KNOTS('',3,(#61109,#61110,#61111,#61112,#61113,
#61114,#61115,#61116,#61117,#61118,#61119,#61120,#61121,#61122,#61123,#61124,
#61125,#61126,#61127,#61128,#61129,#61130,#61131,#61132,#61133,#61134,#61135,
#61136,#61137,#61138,#61139,#61140,#61141,#61142,#61143,#61144,#61145,#61146,
#61147,#61148,#61149,#61150,#61151,#61152,#61153,#61154,#61155,#61156,#61157,
#61158,#61159,#61160,#61161,#61162,#61163,#61164,#61165,#61166,#61167,#61168,
#61169,#61170,#61171,#61172,#61173,#61174,#61175,#61176,#61177,#61178,#61179,
#61180,#61181,#61182,#61183,#61184,#61185,#61186,#61187,#61188,#61189,#61190,
#61191,#61192,#61193,#61194,#61195,#61196,#61197,#61198,#61199,#61200,#61201,
#61202,#61203,#61204,#61205,#61206,#61207,#61208,#61209,#61210,#61211,#61212,
#61213,#61214,#61215,#61216,#61217,#61218,#61219,#61220,#61221,#61222,#61223,
#61224,#61225,#61226,#61227,#61228,#61229,#61230,#61231,#61232),
 .UNSPECIFIED.,.F.,.F.,(4,3,3,3,3,3,3,3,3,3,3,3,3,3,3,3,3,3,3,3,3,3,3,3,
3,3,3,3,3,3,3,3,3,3,3,3,3,3,3,3,3,4),(112.181790913379,112.280032816134,
112.37828191992,112.476633696113,112.575038433759,112.673614612974,112.749405680676,
112.84800380568,112.946461588456,113.046684156229,113.144963713957,113.243210293031,
113.341453376069,113.443150564711,113.54153497813,113.644888554384,113.748242130638,
113.846840255642,113.945298038418,114.045520606191,114.143800163919,114.242046742992,
114.340289826031,114.441987014673,114.540371428091,114.643725004345,114.747078580599,
114.845676705603,114.944134488379,115.044357056152,115.14263661388,115.240883192954,
115.339126275992,115.440823464634,115.539207878053,115.642561454307,115.745915030561,
115.84988875933,115.953561696348,116.057054365165,116.160309146372,116.238928182547),
 .UNSPECIFIED.);
#644=B_SPLINE_CURVE_WITH_KNOTS('',3,(#61233,#61234,#61235,#61236,#61237,
#61238,#61239,#61240,#61241,#61242,#61243,#61244,#61245,#61246,#61247,#61248,
#61249,#61250,#61251,#61252,#61253,#61254,#61255,#61256,#61257,#61258,#61259,
#61260,#61261,#61262,#61263,#61264,#61265,#61266,#61267,#61268,#61269,#61270,
#61271,#61272,#61273,#61274,#61275,#61276,#61277,#61278,#61279,#61280,#61281,
#61282,#61283,#61284,#61285,#61286,#61287,#61288,#61289,#61290,#61291,#61292,
#61293,#61294,#61295,#61296,#61297,#61298,#61299,#61300,#61301,#61302),
 .UNSPECIFIED.,.F.,.F.,(4,3,3,3,3,3,3,3,3,3,3,3,3,3,3,3,3,3,3,3,3,3,3,4),
(116.238928182823,116.341566510357,116.44447107289,116.547509821617,116.650828963887,
116.744751480523,116.843349605527,116.941807388303,117.042029956076,117.140309513804,
117.238556092878,117.336799175916,117.438496364558,117.536880777977,117.640234354231,
117.743587930485,117.842162082218,117.940606624241,118.038951269663,118.137225626956,
118.235476585645,118.33371461238,118.431998836531,118.464214588977),
 .UNSPECIFIED.);
#645=B_SPLINE_CURVE_WITH_KNOTS('',3,(#61304,#61305,#61306,#61307,#61308,
#61309,#61310,#61311,#61312,#61313,#61314,#61315,#61316,#61317,#61318,#61319,
#61320,#61321,#61322,#61323,#61324,#61325,#61326,#61327,#61328,#61329,#61330,
#61331,#61332,#61333,#61334,#61335,#61336,#61337,#61338,#61339,#61340,#61341,
#61342,#61343,#61344,#61345,#61346,#61347,#61348,#61349,#61350,#61351,#61352,
#61353,#61354,#61355,#61356,#61357,#61358,#61359,#61360,#61361,#61362,#61363,
#61364,#61365,#61366,#61367,#61368,#61369,#61370,#61371,#61372,#61373),
 .UNSPECIFIED.,.F.,.F.,(4,3,3,3,3,3,3,3,3,3,3,3,3,3,3,3,3,3,3,3,3,3,3,4),
(116.238928182823,116.279944748004,116.378542873008,116.477000655784,116.577223223557,
116.675502781285,116.773749360358,116.871992443397,116.973689632039,117.072074045458,
117.175427621712,117.278781197966,117.37737932297,117.475837105746,117.576059673519,
117.674339231247,117.77258581032,117.870828893359,117.972526082001,118.07091049542,
118.174264071673,118.277617647927,118.37618931384,118.465360130437),
 .UNSPECIFIED.);
#646=B_SPLINE_CURVE_WITH_KNOTS('',3,(#61374,#61375,#61376,#61377,#61378,
#61379,#61380,#61381),.UNSPECIFIED.,.F.,.F.,(4,1,1,1,1,4),(112.180986309197,
112.284598948156,113.283435398118,114.28227184808,115.281108298042,116.238922797716),
 .UNSPECIFIED.);
#647=B_SPLINE_CURVE_WITH_KNOTS('',3,(#61387,#61388,#61389,#61390,#61391,
#61392,#61393,#61394,#61395,#61396,#61397,#61398,#61399,#61400,#61401,#61402,
#61403,#61404,#61405,#61406,#61407,#61408,#61409,#61410,#61411,#61412,#61413,
#61414,#61415,#61416,#61417,#61418,#61419,#61420,#61421,#61422,#61423,#61424,
#61425,#61426,#61427,#61428,#61429,#61430,#61431,#61432,#61433,#61434,#61435,
#61436,#61437,#61438,#61439,#61440,#61441,#61442,#61443,#61444,#61445,#61446,
#61447,#61448,#61449,#61450,#61451,#61452,#61453,#61454,#61455,#61456,#61457,
#61458,#61459,#61460,#61461,#61462,#61463,#61464,#61465,#61466,#61467,#61468,
#61469,#61470,#61471,#61472,#61473,#61474,#61475,#61476,#61477,#61478,#61479,
#61480,#61481,#61482,#61483,#61484,#61485,#61486,#61487,#61488,#61489,#61490,
#61491,#61492,#61493,#61494,#61495,#61496,#61497,#61498,#61499,#61500,#61501,
#61502,#61503,#61504,#61505,#61506,#61507,#61508,#61509,#61510),
 .UNSPECIFIED.,.F.,.F.,(4,3,3,3,3,3,3,3,3,3,3,3,3,3,3,3,3,3,3,3,3,3,3,3,
3,3,3,3,3,3,3,3,3,3,3,3,3,3,3,3,3,4),(105.898938909624,105.997345956639,
106.095658465059,106.193920742369,106.292162290793,106.390412584537,106.488766476771,
106.58717471803,106.685752797487,106.756386980905,106.854985105909,106.953442888685,
107.053665456458,107.151945014186,107.250191593259,107.348434676298,107.45013186494,
107.548516278359,107.651869854612,107.755223430866,107.85382155587,107.952279338646,
108.052501906419,108.150781464147,108.24902804322,108.347271126259,108.448968314901,
108.54735272832,108.650706304574,108.754059880828,108.852658005832,108.951115788609,
109.051338356381,109.149617914109,109.247864493183,109.346107576221,109.447804764864,
109.546189178282,109.649542754536,109.75289633079,109.893212936346,109.955742875643),
 .UNSPECIFIED.);
#648=B_SPLINE_CURVE_WITH_KNOTS('',3,(#61511,#61512,#61513,#61514,#61515,
#61516,#61517,#61518,#61519,#61520,#61521,#61522,#61523,#61524,#61525,#61526,
#61527,#61528,#61529,#61530,#61531,#61532,#61533,#61534,#61535,#61536,#61537,
#61538,#61539,#61540,#61541,#61542,#61543,#61544,#61545,#61546,#61547,#61548,
#61549,#61550,#61551,#61552,#61553,#61554,#61555,#61556,#61557,#61558,#61559,
#61560,#61561,#61562,#61563,#61564,#61565,#61566,#61567,#61568,#61569,#61570,
#61571,#61572,#61573,#61574,#61575,#61576,#61577,#61578,#61579,#61580,#61581,
#61582,#61583),.UNSPECIFIED.,.F.,.F.,(4,3,3,3,3,3,3,3,3,3,3,3,3,3,3,3,3,
3,3,3,3,3,3,3,4),(109.955742875951,110.055241614051,110.152151423466,110.249014842069,
110.345862894414,110.447330365998,110.544300028994,110.641334438528,110.738518045248,
110.751732780752,110.850330905756,110.948788688532,111.049011256305,111.147290814033,
111.245537393107,111.343780476145,111.445477664787,111.543862078206,111.64721565446,
111.750569230714,111.849176820417,111.947618966289,112.045965736414,112.144240689696,
112.181790913379),.UNSPECIFIED.);
#649=B_SPLINE_CURVE_WITH_KNOTS('',3,(#61585,#61586,#61587,#61588,#61589,
#61590),.UNSPECIFIED.,.F.,.F.,(4,1,1,4),(109.955750010575,110.286926048232,
111.285762498194,112.180986309197),.UNSPECIFIED.);
#650=B_SPLINE_CURVE_WITH_KNOTS('',3,(#61591,#61592,#61593,#61594,#61595,
#61596,#61597,#61598,#61599,#61600,#61601,#61602,#61603,#61604,#61605,#61606,
#61607,#61608,#61609,#61610,#61611,#61612,#61613,#61614,#61615,#61616,#61617,
#61618,#61619,#61620,#61621,#61622,#61623,#61624,#61625,#61626,#61627,#61628,
#61629,#61630,#61631,#61632,#61633,#61634,#61635,#61636,#61637,#61638,#61639,
#61640,#61641,#61642,#61643,#61644,#61645,#61646,#61647,#61648,#61649,#61650,
#61651,#61652,#61653,#61654,#61655,#61656,#61657,#61658,#61659,#61660,#61661,
#61662,#61663,#61664,#61665,#61666,#61667,#61668,#61669,#61670,#61671,#61672,
#61673,#61674,#61675,#61676,#61677,#61678,#61679,#61680,#61681,#61682,#61683,
#61684,#61685,#61686,#61687,#61688,#61689,#61690,#61691,#61692,#61693,#61694,
#61695,#61696,#61697,#61698,#61699,#61700,#61701,#61702,#61703,#61704,#61705,
#61706,#61707,#61708,#61709,#61710,#61711,#61712,#61713,#61714),
 .UNSPECIFIED.,.F.,.F.,(4,3,3,3,3,3,3,3,3,3,3,3,3,3,3,3,3,3,3,3,3,3,3,3,
3,3,3,3,3,3,3,3,3,3,3,3,3,3,3,3,3,4),(105.898082526351,105.996456956859,
106.094847333998,106.193416304684,106.291580248385,106.390178373389,106.488636156165,
106.588858723938,106.687138281666,106.78538486074,106.883627943778,106.98532513242,
107.083709545839,107.187063122093,107.290416698347,107.389014823351,107.487472606127,
107.5876951739,107.685974731628,107.784221310702,107.88246439374,107.984161582382,
108.082545995801,108.185899572055,108.289253148309,108.387851273313,108.48630905609,
108.586531623862,108.68481118159,108.783057760664,108.881300843702,108.982998032344,
109.081382445763,109.184736022017,109.288089598271,109.386591328536,109.484956309732,
109.583214317042,109.681399820024,109.779540599734,109.877698313765,109.955742875643),
 .UNSPECIFIED.);
#651=B_SPLINE_CURVE_WITH_KNOTS('',3,(#61720,#61721,#61722,#61723,#61724,
#61725,#61726,#61727),.UNSPECIFIED.,.F.,.F.,(4,1,1,1,1,4),(99.6144332140862,
99.7645318311714,100.763368281133,101.762204731095,102.761041181057,103.672548858805),
 .UNSPECIFIED.);
#652=B_SPLINE_CURVE_WITH_KNOTS('',3,(#61728,#61729,#61730,#61731,#61732,
#61733,#61734,#61735,#61736,#61737,#61738,#61739,#61740,#61741,#61742,#61743,
#61744,#61745,#61746,#61747,#61748,#61749,#61750,#61751,#61752,#61753,#61754,
#61755,#61756,#61757,#61758,#61759,#61760,#61761,#61762,#61763,#61764,#61765,
#61766,#61767,#61768,#61769,#61770,#61771,#61772,#61773,#61774,#61775,#61776,
#61777,#61778,#61779,#61780,#61781,#61782,#61783,#61784,#61785,#61786,#61787,
#61788,#61789,#61790,#61791,#61792,#61793,#61794,#61795,#61796,#61797),
 .UNSPECIFIED.,.F.,.F.,(4,3,3,3,3,3,3,3,3,3,3,3,3,3,3,3,3,3,3,3,3,3,3,4),
(103.672557568463,103.759877631019,103.858475756023,103.956933538799,104.057156106572,
104.1554356643,104.253682243374,104.351925326412,104.453622515054,104.552006928473,
104.655360504727,104.758714080981,104.857312205985,104.955769988762,105.055992556534,
105.154272114262,105.252518693336,105.350761776374,105.452458965017,105.550843378435,
105.654196954689,105.757550530943,105.856140410593,105.898938909624),
 .UNSPECIFIED.);
#653=B_SPLINE_CURVE_WITH_KNOTS('',3,(#61799,#61800,#61801,#61802,#61803,
#61804,#61805,#61806,#61807,#61808,#61809,#61810,#61811,#61812,#61813,#61814,
#61815,#61816,#61817,#61818,#61819,#61820,#61821,#61822,#61823,#61824,#61825,
#61826,#61827,#61828,#61829,#61830,#61831,#61832,#61833,#61834,#61835,#61836,
#61837,#61838,#61839,#61840,#61841,#61842,#61843,#61844,#61845,#61846,#61847,
#61848,#61849,#61850,#61851,#61852,#61853,#61854,#61855,#61856,#61857,#61858,
#61859,#61860,#61861,#61862,#61863,#61864,#61865,#61866,#61867,#61868,#61869,
#61870,#61871),.UNSPECIFIED.,.F.,.F.,(4,3,3,3,3,3,3,3,3,3,3,3,3,3,3,3,3,
3,3,3,3,3,3,3,4),(103.672557568463,103.771601702603,103.870660322484,103.96976131202,
104.06899945985,104.168318657834,104.267812431338,104.293907348461,104.392505473465,
104.490963256241,104.591185824014,104.689465381742,104.787711960816,104.885955043854,
104.987652232496,105.086036645915,105.189390222169,105.292743798423,105.391329160732,
105.489781902013,105.591857058097,105.690131964868,105.788367320327,105.886604354657,
105.898082526351),.UNSPECIFIED.);
#654=B_SPLINE_CURVE_WITH_KNOTS('',3,(#61872,#61873,#61874,#61875,#61876,
#61877,#61878,#61879),.UNSPECIFIED.,.F.,.F.,(4,1,1,1,1,4),(99.616027874956,
100.298561548614,101.297397998576,102.296234448537,103.295070898499,103.672550060316),
 .UNSPECIFIED.);
#655=B_SPLINE_CURVE_WITH_KNOTS('',3,(#61885,#61886,#61887,#61888,#61889,
#61890,#61891,#61892,#61893,#61894,#61895,#61896,#61897,#61898,#61899,#61900,
#61901,#61902,#61903,#61904,#61905,#61906,#61907,#61908,#61909,#61910,#61911,
#61912,#61913,#61914,#61915,#61916,#61917,#61918,#61919,#61920,#61921,#61922,
#61923,#61924,#61925,#61926,#61927,#61928,#61929,#61930,#61931,#61932,#61933,
#61934,#61935,#61936,#61937,#61938,#61939,#61940,#61941,#61942,#61943,#61944,
#61945,#61946,#61947,#61948,#61949,#61950,#61951,#61952,#61953,#61954,#61955,
#61956,#61957,#61958,#61959,#61960,#61961,#61962,#61963,#61964,#61965,#61966,
#61967,#61968,#61969,#61970,#61971,#61972,#61973,#61974,#61975,#61976,#61977,
#61978,#61979,#61980,#61981,#61982,#61983,#61984,#61985,#61986,#61987,#61988,
#61989,#61990,#61991,#61992,#61993,#61994,#61995,#61996,#61997,#61998,#61999,
#62000,#62001,#62002,#62003,#62004,#62005,#62006,#62007,#62008,#62009,#62010,
#62011),.UNSPECIFIED.,.F.,.F.,(4,3,3,3,3,3,3,3,3,3,3,3,3,3,3,3,3,3,3,3,
3,3,3,3,3,3,3,3,3,3,3,3,3,3,3,3,3,3,3,3,3,3,4),(93.3318434365138,93.4301005194132,
93.5284655037585,93.6268914566206,93.7254798312946,93.7715131314001,93.8701112564038,
93.9685690391803,94.068791606953,94.1670711646811,94.2653177437544,94.3635608267929,
94.4652580154352,94.5636424288539,94.666996005108,94.770349581362,94.8689477063657,
94.9674054891425,95.0676280569152,95.1659076146433,95.2641541937166,95.3623972767552,
95.4640944653974,95.5624788788163,95.6658324550701,95.7691860313239,95.8677841563277,
95.9662419391043,96.066464506877,96.1647440646052,96.2629906436784,96.3612337267171,
96.4629309153592,96.5613153287781,96.6646689050319,96.7680224812858,96.8674993725789,
96.9668292609827,97.0660403563899,97.1651524247994,97.2642075332238,97.3632407686269,
97.3893722612837),.UNSPECIFIED.);
#656=B_SPLINE_CURVE_WITH_KNOTS('',3,(#62012,#62013,#62014,#62015,#62016,
#62017),.UNSPECIFIED.,.F.,.F.,(4,1,1,4),(97.3893797693875,97.7668589312476,
98.7656953812095,99.6144332140862),.UNSPECIFIED.);
#657=B_SPLINE_CURVE_WITH_KNOTS('',3,(#62019,#62020,#62021,#62022,#62023,
#62024),.UNSPECIFIED.,.F.,.F.,(4,1,1,4),(97.3893809708947,98.3008886486899,
99.2997250986518,99.616027874956),.UNSPECIFIED.);
#658=B_SPLINE_CURVE_WITH_KNOTS('',3,(#62025,#62026,#62027,#62028,#62029,
#62030,#62031,#62032,#62033,#62034,#62035,#62036,#62037,#62038,#62039,#62040,
#62041,#62042,#62043,#62044,#62045,#62046,#62047,#62048,#62049,#62050,#62051,
#62052,#62053,#62054,#62055,#62056,#62057,#62058,#62059,#62060,#62061,#62062,
#62063,#62064,#62065,#62066,#62067,#62068,#62069,#62070,#62071,#62072,#62073,
#62074,#62075,#62076,#62077,#62078,#62079,#62080,#62081,#62082,#62083,#62084,
#62085,#62086,#62087,#62088,#62089,#62090,#62091,#62092,#62093,#62094,#62095,
#62096,#62097,#62098,#62099,#62100,#62101,#62102,#62103,#62104,#62105,#62106,
#62107,#62108,#62109,#62110,#62111,#62112,#62113,#62114,#62115,#62116,#62117,
#62118,#62119,#62120,#62121,#62122,#62123,#62124,#62125,#62126,#62127,#62128,
#62129,#62130,#62131,#62132,#62133,#62134,#62135,#62136,#62137,#62138,#62139,
#62140,#62141,#62142,#62143,#62144,#62145,#62146,#62147,#62148),
 .UNSPECIFIED.,.F.,.F.,(4,3,3,3,3,3,3,3,3,3,3,3,3,3,3,3,3,3,3,3,3,3,3,3,
3,3,3,3,3,3,3,3,3,3,3,3,3,3,3,3,3,4),(93.3321733081382,93.4307320543271,
93.5291589455774,93.62748337466,93.7257523655947,93.8239954283074,93.9222420400156,
94.0205891010754,94.1189858425587,94.2175578841727,94.3055428488424,94.4041409738461,
94.5025987566228,94.6028213243955,94.7011008821237,94.7993474611971,94.8975905442356,
94.9992877328777,95.0976721462965,95.2010257225504,95.3043792988043,95.402977423808,
95.5014352065847,95.6016577743574,95.6999373320856,95.798183911159,95.8964269941975,
95.9981241828397,96.0965085962585,96.1998621725124,96.3032157487662,96.4018138737699,
96.5002716565467,96.6004942243194,96.6987737820475,96.7970203611209,96.8952634441594,
96.9969606328015,97.0953450462203,97.1986986224742,97.302052198728,97.3893722612837),
 .UNSPECIFIED.);
#659=B_SPLINE_CURVE_WITH_KNOTS('',3,(#62154,#62155,#62156,#62157,#62158,
#62159,#62160,#62161),.UNSPECIFIED.,.F.,.F.,(4,1,1,1,1,4),(87.0497429142915,
87.7784944316289,88.7773308815908,89.7761673315526,90.7750037815145,91.1061798192275),
 .UNSPECIFIED.);
#660=B_SPLINE_CURVE_WITH_KNOTS('',3,(#62162,#62163,#62164,#62165,#62166,
#62167,#62168,#62169,#62170,#62171,#62172,#62173,#62174,#62175,#62176,#62177,
#62178,#62179,#62180,#62181,#62182,#62183,#62184,#62185,#62186,#62187,#62188,
#62189,#62190,#62191,#62192,#62193,#62194,#62195,#62196,#62197,#62198,#62199,
#62200,#62201,#62202,#62203,#62204,#62205,#62206,#62207,#62208,#62209,#62210,
#62211,#62212,#62213,#62214,#62215,#62216,#62217,#62218,#62219,#62220,#62221,
#62222,#62223,#62224,#62225,#62226,#62227,#62228,#62229,#62230,#62231),
 .UNSPECIFIED.,.F.,.F.,(4,3,3,3,3,3,3,3,3,3,3,3,3,3,3,3,3,3,3,3,3,3,3,4),
(91.1061869541041,91.204341964477,91.3024795334308,91.400629164884,91.4988897541857,
91.5972075103079,91.6957053368615,91.7738402314764,91.8724383564801,91.9708961392567,
92.0711187070294,92.1693982647576,92.267644843831,92.3658879268695,92.4675851155117,
92.5659695289305,92.6693231051844,92.7726766814383,92.871267317254,92.9697241251268,
93.0680663331376,93.1663410384432,93.2645927043616,93.3318434365138),
 .UNSPECIFIED.);
#661=B_SPLINE_CURVE_WITH_KNOTS('',3,(#62233,#62234,#62235,#62236,#62237,
#62238,#62239,#62240,#62241,#62242,#62243,#62244,#62245,#62246,#62247,#62248,
#62249,#62250,#62251,#62252,#62253,#62254,#62255,#62256,#62257,#62258,#62259,
#62260,#62261,#62262,#62263,#62264,#62265,#62266,#62267,#62268,#62269,#62270,
#62271,#62272,#62273,#62274,#62275,#62276,#62277,#62278,#62279,#62280,#62281,
#62282,#62283,#62284,#62285,#62286,#62287,#62288,#62289,#62290,#62291,#62292,
#62293,#62294,#62295,#62296,#62297,#62298,#62299,#62300,#62301,#62302),
 .UNSPECIFIED.,.F.,.F.,(4,3,3,3,3,3,3,3,3,3,3,3,3,3,3,3,3,3,3,3,3,3,3,4),
(91.1061869541041,91.2465035596771,91.3090334989568,91.4076316239605,91.5060894067374,
91.60631197451,91.7045915322382,91.8028381113116,91.9010811943501,92.0027783829923,
92.101162796411,92.2045163726649,92.3078699489187,92.4064680739224,92.5049258566991,
92.6051484244718,92.7034279822,92.8016745612733,92.8999176443118,93.001614832954,
93.0999992463728,93.2033528226267,93.3067063988806,93.3321733081382),
 .UNSPECIFIED.);
#662=B_SPLINE_CURVE_WITH_KNOTS('',3,(#62303,#62304,#62305,#62306,#62307,
#62308,#62309,#62310,#62311,#62312,#62313,#62314,#62315,#62316,#62317,#62318,
#62319,#62320,#62321,#62322,#62323,#62324,#62325,#62326,#62327,#62328,#62329,
#62330,#62331,#62332,#62333,#62334,#62335,#62336,#62337,#62338,#62339,#62340,
#62341,#62342,#62343,#62344,#62345,#62346,#62347,#62348,#62349,#62350,#62351,
#62352,#62353,#62354,#62355,#62356,#62357,#62358,#62359,#62360,#62361,#62362,
#62363,#62364,#62365,#62366,#62367,#62368,#62369,#62370,#62371,#62372,#62373,
#62374,#62375,#62376,#62377,#62378,#62379,#62380,#62381,#62382,#62383,#62384,
#62385,#62386,#62387,#62388,#62389,#62390,#62391,#62392,#62393,#62394,#62395,
#62396,#62397,#62398,#62399,#62400,#62401,#62402,#62403,#62404,#62405,#62406,
#62407,#62408,#62409,#62410,#62411,#62412,#62413,#62414,#62415,#62416,#62417,
#62418,#62419,#62420,#62421,#62422,#62423,#62424,#62425,#62426,#62427,#62428,
#62429),.UNSPECIFIED.,.F.,.F.,(4,3,3,3,3,3,3,3,3,3,3,3,3,3,3,3,3,3,3,3,
3,3,3,3,3,3,3,3,3,3,3,3,3,3,3,3,3,3,3,3,3,3,4),(87.0482730518095,87.1466828155122,
87.2452617360055,87.3136876991093,87.412285824113,87.5107436068898,87.6109661746624,
87.7092457323906,87.807492311464,87.9057353945025,88.0074325831446,88.1058169965635,
88.2091705728173,88.3125241490712,88.4111222740749,88.5095800568516,88.6098026246243,
88.7080821823525,88.8063287614259,88.9045718444644,89.0062690331065,89.1046534465253,
89.2080070227792,89.3113605990331,89.4099587240368,89.5084165068135,89.6086390745861,
89.7069186323143,89.8051652113877,89.9034082944262,90.0051054830683,90.1034898964871,
90.206843472741,90.3101970489949,90.409695787095,90.5067185530535,90.6036495481491,
90.7005198981798,90.8019366620839,90.8988156754796,90.9957205549586,91.0927209416411,
91.1061869537961),.UNSPECIFIED.);
#663=B_SPLINE_CURVE_WITH_KNOTS('',3,(#62435,#62436,#62437,#62438,#62439,
#62440,#62441,#62442,#62443,#62444,#62445,#62446,#62447,#62448,#62449,#62450,
#62451,#62452,#62453,#62454,#62455,#62456,#62457,#62458,#62459,#62460,#62461,
#62462,#62463,#62464,#62465,#62466,#62467,#62468,#62469,#62470,#62471,#62472,
#62473,#62474,#62475,#62476,#62477,#62478,#62479,#62480,#62481,#62482,#62483,
#62484,#62485,#62486,#62487,#62488,#62489,#62490,#62491,#62492,#62493,#62494,
#62495,#62496,#62497,#62498,#62499,#62500,#62501,#62502,#62503,#62504,#62505,
#62506,#62507,#62508,#62509,#62510,#62511,#62512,#62513,#62514,#62515,#62516,
#62517,#62518,#62519,#62520,#62521,#62522,#62523,#62524,#62525,#62526,#62527,
#62528,#62529,#62530,#62531,#62532,#62533,#62534,#62535,#62536,#62537,#62538,
#62539,#62540,#62541,#62542,#62543,#62544,#62545,#62546,#62547,#62548,#62549,
#62550,#62551,#62552,#62553,#62554,#62555,#62556,#62557,#62558,#62559,#62560,
#62561),.UNSPECIFIED.,.F.,.F.,(4,3,3,3,3,3,3,3,3,3,3,3,3,3,3,3,3,3,3,3,
3,3,3,3,3,3,3,3,3,3,3,3,3,3,3,3,3,3,3,3,3,3,4),(80.7655329441315,80.7866392818958,
80.8852374068995,80.9836951896762,81.0839177574489,81.182197315177,81.2804438942504,
81.3786869772889,81.4803841659311,81.5787685793499,81.6821221556038,81.7854757318576,
81.8840738568613,81.9825316396381,82.0827542074107,82.1810337651388,82.2792803442122,
82.3775234272507,82.4792206158929,82.5776050293117,82.6809586055656,82.7843121818195,
82.8829103068232,82.9813680896,83.0815906573726,83.1798702151008,83.2781167941742,
83.3763598772127,83.4780570658549,83.5764414792737,83.6797950555275,83.7831486317814,
83.8817467567851,83.9802045395617,84.0804271073344,84.1787066650625,84.2769532441359,
84.3751963271743,84.4768935158166,84.5752779292353,84.6786315054893,84.7819850817433,
84.8230016469246),.UNSPECIFIED.);
#664=B_SPLINE_CURVE_WITH_KNOTS('',3,(#62562,#62563,#62564,#62565,#62566,
#62567),.UNSPECIFIED.,.F.,.F.,(4,1,1,4),(84.8230070320566,85.7808215317051,
86.779657981667,87.0497429142915),.UNSPECIFIED.);
#665=B_SPLINE_CURVE_WITH_KNOTS('',3,(#62569,#62570,#62571,#62572,#62573,
#62574,#62575,#62576,#62577,#62578,#62579,#62580,#62581,#62582,#62583,#62584,
#62585,#62586,#62587,#62588,#62589,#62590,#62591,#62592,#62593,#62594,#62595,
#62596,#62597,#62598,#62599,#62600,#62601,#62602,#62603,#62604,#62605,#62606,
#62607,#62608,#62609,#62610,#62611,#62612,#62613,#62614,#62615,#62616,#62617,
#62618,#62619,#62620,#62621,#62622,#62623,#62624,#62625,#62626,#62627,#62628,
#62629,#62630,#62631,#62632,#62633,#62634,#62635,#62636,#62637,#62638),
 .UNSPECIFIED.,.F.,.F.,(4,3,3,3,3,3,3,3,3,3,3,3,3,3,3,3,3,3,3,3,3,3,3,4),
(84.8230016472006,84.9261861619506,85.0296647966982,85.1332945907094,85.2372126194226,
85.3160147991856,85.4146129241893,85.5130707069661,85.6132932747388,85.7115728324669,
85.8098194115403,85.9080624945788,86.0097596832209,86.1081440966397,86.2114976728936,
86.3148512491474,86.4134243290395,86.5118681332278,86.6102123732684,86.7084866565498,
86.8067399239169,86.9049803913479,87.0032727094468,87.0482730518095),
 .UNSPECIFIED.);
#666=B_SPLINE_CURVE_WITH_KNOTS('',3,(#62639,#62640,#62641,#62642,#62643,
#62644,#62645,#62646,#62647,#62648,#62649,#62650,#62651,#62652,#62653,#62654,
#62655,#62656,#62657,#62658,#62659,#62660,#62661,#62662,#62663,#62664,#62665,
#62666,#62667,#62668,#62669,#62670,#62671,#62672,#62673,#62674,#62675,#62676,
#62677,#62678,#62679,#62680,#62681,#62682,#62683,#62684,#62685,#62686,#62687,
#62688,#62689,#62690,#62691,#62692,#62693,#62694,#62695,#62696,#62697,#62698,
#62699,#62700,#62701,#62702,#62703,#62704,#62705,#62706,#62707,#62708,#62709,
#62710,#62711,#62712,#62713,#62714,#62715,#62716,#62717,#62718,#62719,#62720,
#62721,#62722,#62723,#62724,#62725,#62726,#62727,#62728,#62729,#62730,#62731,
#62732,#62733,#62734,#62735,#62736,#62737,#62738,#62739,#62740,#62741,#62742,
#62743,#62744,#62745,#62746,#62747,#62748,#62749,#62750,#62751,#62752,#62753,
#62754,#62755,#62756,#62757,#62758,#62759,#62760,#62761,#62762),
 .UNSPECIFIED.,.F.,.F.,(4,3,3,3,3,3,3,3,3,3,3,3,3,3,3,3,3,3,3,3,3,3,3,3,
3,3,3,3,3,3,3,3,3,3,3,3,3,3,3,3,3,4),(80.7658264624535,80.8640676348504,
80.9623198392987,81.0606769983247,81.1590905612312,81.2576716189549,81.3206689993381,
81.4192671243418,81.5177249071187,81.6179474748913,81.7162270326195,81.8144736116928,
81.9127166947314,82.0144138833735,82.1127982967923,82.2161518730461,82.3195054492999,
82.4181035743036,82.5165613570802,82.6167839248529,82.7150634825809,82.8133100616542,
82.9115531446927,83.013250333335,83.1116347467538,83.2149883230078,83.3183418992618,
83.4169400242654,83.5153978070423,83.615620374815,83.7138999325431,83.8121465116164,
83.9103895946548,84.0120867832971,84.1104711967158,84.2138247729698,84.3171783492237,
84.4205578302504,84.5236543867486,84.6265834813177,84.7292989065991,84.8230016469246),
 .UNSPECIFIED.);
#667=B_SPLINE_CURVE_WITH_KNOTS('',3,(#62768,#62769,#62770,#62771,#62772,
#62773,#62774,#62775),.UNSPECIFIED.,.F.,.F.,(4,1,1,1,1,4),(74.4816441096174,
74.7936205821245,75.7924570320864,76.7912934820483,77.7901299320101,78.539816339745),
 .UNSPECIFIED.);
#668=B_SPLINE_CURVE_WITH_KNOTS('',3,(#62776,#62777,#62778,#62779,#62780,
#62781,#62782,#62783,#62784,#62785,#62786,#62787,#62788,#62789,#62790,#62791,
#62792,#62793,#62794,#62795,#62796,#62797,#62798,#62799,#62800,#62801,#62802,
#62803,#62804,#62805,#62806,#62807,#62808,#62809,#62810,#62811,#62812,#62813,
#62814,#62815,#62816,#62817,#62818,#62819,#62820,#62821,#62822,#62823,#62824,
#62825,#62826,#62827,#62828,#62829,#62830,#62831,#62832,#62833,#62834,#62835,
#62836,#62837,#62838,#62839,#62840,#62841,#62842),.UNSPECIFIED.,.F.,.F.,
(4,3,3,3,3,3,3,3,3,3,3,3,3,3,3,3,3,3,3,3,3,3,4),(78.5398164398063,78.6677108218491,
78.788966381972,78.8875645069757,78.9860222897523,79.086244857525,79.1845244152532,
79.2827709943266,79.3810140773651,79.4827112660073,79.5810956794261,79.68444925568,
79.7878028319339,79.8864023576712,79.9848611556908,80.0832042043534,80.1814836418347,
80.2797289912669,80.3779697355283,80.4762993937657,80.5746716764509,80.673210932794,
80.7655329441315),.UNSPECIFIED.);
#669=B_SPLINE_CURVE_WITH_KNOTS('',3,(#62844,#62845,#62846,#62847,#62848,
#62849,#62850,#62851,#62852,#62853,#62854,#62855,#62856,#62857,#62858,#62859,
#62860,#62861,#62862,#62863,#62864,#62865,#62866,#62867,#62868,#62869,#62870,
#62871,#62872,#62873,#62874,#62875,#62876,#62877,#62878,#62879,#62880,#62881,
#62882,#62883,#62884,#62885,#62886,#62887,#62888,#62889,#62890,#62891,#62892,
#62893,#62894,#62895,#62896,#62897,#62898,#62899,#62900,#62901,#62902,#62903,
#62904,#62905,#62906,#62907,#62908,#62909,#62910,#62911,#62912,#62913),
 .UNSPECIFIED.,.F.,.F.,(4,3,3,3,3,3,3,3,3,3,3,3,3,3,3,3,3,3,3,3,3,3,3,4),
(78.539816339745,78.6377138097037,78.7346673304386,78.8315786913982,78.9284788661298,
79.0271081744509,79.1241353185132,79.2235657089638,79.3229960994143,79.421594224418,
79.5200520071948,79.6202745749675,79.7185541326956,79.8168007117689,79.9150437948075,
80.0167409834497,80.1151253968685,80.2184789731223,80.3218325493762,80.420438292131,
80.5188792313176,80.617224929138,80.7155010605394,80.7658264624535),
 .UNSPECIFIED.);
#670=B_SPLINE_CURVE_WITH_KNOTS('',3,(#62914,#62915,#62916,#62917,#62918,
#62919,#62920,#62921),.UNSPECIFIED.,.F.,.F.,(4,1,1,1,1,4),(74.4832630428072,
75.3276502995668,76.3264867495287,77.3253231994906,78.3241596494524,78.539816339745),
 .UNSPECIFIED.);
#671=B_SPLINE_CURVE_WITH_KNOTS('',3,(#62927,#62928,#62929,#62930,#62931,
#62932,#62933,#62934,#62935,#62936,#62937,#62938,#62939,#62940,#62941,#62942,
#62943,#62944,#62945,#62946,#62947,#62948,#62949,#62950,#62951,#62952,#62953,
#62954,#62955,#62956,#62957,#62958,#62959,#62960,#62961,#62962,#62963,#62964,
#62965,#62966,#62967,#62968,#62969,#62970,#62971,#62972,#62973,#62974,#62975,
#62976,#62977,#62978,#62979,#62980,#62981,#62982,#62983,#62984,#62985,#62986,
#62987,#62988,#62989,#62990,#62991,#62992,#62993,#62994,#62995,#62996,#62997,
#62998,#62999,#63000,#63001,#63002,#63003,#63004,#63005,#63006,#63007,#63008,
#63009,#63010,#63011,#63012,#63013,#63014,#63015,#63016,#63017,#63018,#63019,
#63020,#63021,#63022,#63023,#63024,#63025,#63026,#63027,#63028,#63029,#63030,
#63031,#63032,#63033,#63034,#63035,#63036,#63037,#63038,#63039,#63040,#63041,
#63042,#63043,#63044,#63045,#63046,#63047,#63048,#63049,#63050),
 .UNSPECIFIED.,.F.,.F.,(4,3,3,3,3,3,3,3,3,3,3,3,3,3,3,3,3,3,3,3,3,3,3,3,
3,3,3,3,3,3,3,3,3,3,3,3,3,3,3,3,3,4),(68.1995885751602,68.2978347417454,
68.3960780917011,68.4972090393642,68.5955944498561,68.6980981661047,68.8006018823533,
68.8992000073569,68.9976577901337,69.0978803579063,69.1961599156345,69.2944064947079,
69.3926495777462,69.4943467663884,69.5927311798072,69.6960847560611,69.7994383323151,
69.8980364573188,69.9964942400957,70.0967168078684,70.1949963655966,70.2932429446699,
70.3914860277088,70.4931832163508,70.5915676297697,70.6949212060233,70.798274782277,
70.8968729072808,70.9953306900575,71.0955532578301,71.1938328155584,71.2920793946318,
71.3903224776704,71.4920196663125,71.5904040797312,71.6937576559851,71.7971112322389,
71.9028340905518,72.0081993817383,72.1133399321502,72.2181701837247,72.2566308185806),
 .UNSPECIFIED.);
#672=B_SPLINE_CURVE_WITH_KNOTS('',3,(#63051,#63052,#63053,#63054,#63055,
#63056),.UNSPECIFIED.,.F.,.F.,(4,1,1,4),(72.2566310325654,72.7959476822008,
73.7947841321626,74.4816441096174),.UNSPECIFIED.);
#673=B_SPLINE_CURVE_WITH_KNOTS('',3,(#63058,#63059,#63060,#63061,#63062,
#63063,#63064),.UNSPECIFIED.,.F.,.F.,(4,1,1,1,4),(72.2566310325654,72.3311409496812,
73.3299773996431,74.3288138496049,74.4832630428072),.UNSPECIFIED.);
#674=B_SPLINE_CURVE_WITH_KNOTS('',3,(#63065,#63066,#63067,#63068,#63069,
#63070,#63071,#63072,#63073,#63074,#63075,#63076,#63077,#63078,#63079,#63080,
#63081,#63082,#63083,#63084,#63085,#63086,#63087,#63088,#63089,#63090,#63091,
#63092,#63093,#63094,#63095,#63096,#63097,#63098,#63099,#63100,#63101,#63102,
#63103,#63104,#63105,#63106,#63107,#63108,#63109,#63110,#63111,#63112,#63113,
#63114,#63115,#63116,#63117,#63118,#63119,#63120,#63121,#63122,#63123,#63124,
#63125,#63126,#63127,#63128,#63129,#63130,#63131,#63132,#63133,#63134,#63135,
#63136,#63137,#63138,#63139,#63140,#63141,#63142,#63143,#63144,#63145,#63146,
#63147,#63148,#63149,#63150,#63151,#63152,#63153,#63154,#63155,#63156,#63157,
#63158,#63159,#63160,#63161,#63162,#63163,#63164,#63165,#63166,#63167,#63168,
#63169,#63170,#63171,#63172,#63173,#63174,#63175,#63176,#63177,#63178,#63179,
#63180,#63181,#63182,#63183,#63184,#63185,#63186,#63187,#63188,#63189,#63190,
#63191),.UNSPECIFIED.,.F.,.F.,(4,3,3,3,3,3,3,3,3,3,3,3,3,3,3,3,3,3,3,3,
3,3,3,3,3,3,3,3,3,3,3,3,3,3,3,3,3,3,3,3,3,3,4),(68.1987514894476,68.2973434467588,
68.3357951498337,68.4343932748374,68.5328510576141,68.6330736253868,68.731353183115,
68.8295997621883,68.9278428452268,69.029540033869,69.1279244472878,69.2312780235417,
69.3346315997956,69.4332297247993,69.5316875075761,69.6319100753487,69.7301896330769,
69.8284362121503,69.9266792951887,70.0283764838309,70.1267608972497,70.2301144735036,
70.3334680497574,70.4320661747611,70.5305239575378,70.6307465253105,70.7290260830387,
70.8272726621121,70.9255157451505,71.0272129337927,71.1255973472115,71.2289509234654,
71.3323044997193,71.4298807240689,71.5273176349422,71.6246428433671,71.7219081150621,
71.8191441424517,71.9163815796695,72.013708783522,72.1110862397604,72.2086145464311,
72.2566310325654),.UNSPECIFIED.);
#675=B_SPLINE_CURVE_WITH_KNOTS('',3,(#63197,#63198,#63199,#63200,#63201,
#63202,#63203,#63204),.UNSPECIFIED.,.F.,.F.,(4,1,1,1,1,4),(61.9167164720863,
62.807583182582,63.8064196325439,64.8052560825058,65.8040925324676,65.9734457253857),
 .UNSPECIFIED.);
#676=B_SPLINE_CURVE_WITH_KNOTS('',3,(#63205,#63206,#63207,#63208,#63209,
#63210,#63211,#63212,#63213,#63214,#63215,#63216,#63217,#63218,#63219,#63220,
#63221,#63222,#63223,#63224,#63225,#63226,#63227,#63228,#63229,#63230,#63231,
#63232,#63233,#63234,#63235,#63236,#63237,#63238,#63239,#63240,#63241,#63242,
#63243,#63244,#63245,#63246,#63247,#63248,#63249,#63250,#63251,#63252,#63253,
#63254,#63255,#63256,#63257,#63258,#63259,#63260,#63261,#63262,#63263,#63264,
#63265,#63266,#63267,#63268,#63269,#63270,#63271,#63272,#63273,#63274),
 .UNSPECIFIED.,.F.,.F.,(4,3,3,3,3,3,3,3,3,3,3,3,3,3,3,3,3,3,3,3,3,3,3,4),
(65.9734457253857,66.0704340596178,66.1673127975358,66.264132888756,66.360925426791,
66.4577214670338,66.5546134226801,66.6515579893416,66.7486626585399,66.8029289824295,
66.9015271074332,66.99998489021,67.1002074579827,67.1984870157108,67.2967335947842,
67.3949766778227,67.4966738664649,67.5950582798838,67.6984118561376,67.8017654323914,
67.9012212180836,67.9996662359346,68.0996274055474,68.1995885751602),
 .UNSPECIFIED.);
#677=B_SPLINE_CURVE_WITH_KNOTS('',3,(#63276,#63277,#63278,#63279,#63280,
#63281,#63282,#63283,#63284,#63285,#63286,#63287,#63288,#63289,#63290,#63291,
#63292,#63293,#63294,#63295,#63296,#63297,#63298,#63299,#63300,#63301,#63302,
#63303,#63304,#63305,#63306,#63307,#63308,#63309,#63310,#63311,#63312,#63313,
#63314,#63315,#63316,#63317,#63318,#63319,#63320,#63321,#63322,#63323,#63324,
#63325,#63326,#63327,#63328,#63329,#63330,#63331,#63332,#63333,#63334,#63335,
#63336,#63337,#63338,#63339,#63340,#63341,#63342,#63343,#63344,#63345),
 .UNSPECIFIED.,.F.,.F.,(4,3,3,3,3,3,3,3,3,3,3,3,3,3,3,3,3,3,3,3,3,3,3,4),
(65.9734457256204,66.084879805074,66.1968635637049,66.3094957826842,66.3381222499099,
66.4367203749136,66.5351781576905,66.6354007254632,66.7336802831913,66.8319268622647,
66.9301699453032,67.0318671339454,67.1302515473642,67.233605123618,67.3369586998718,
67.4355663370611,67.534004594347,67.632346634809,67.7306220560113,67.8288603843819,
67.9271329658687,68.0254205103534,68.1238183934725,68.1987514894476),
 .UNSPECIFIED.);
#678=B_SPLINE_CURVE_WITH_KNOTS('',3,(#63346,#63347,#63348,#63349,#63350,
#63351,#63352,#63353,#63354,#63355,#63356,#63357,#63358,#63359,#63360,#63361,
#63362,#63363,#63364,#63365,#63366,#63367,#63368,#63369,#63370,#63371,#63372,
#63373,#63374,#63375,#63376,#63377,#63378,#63379,#63380,#63381,#63382,#63383,
#63384,#63385,#63386,#63387,#63388,#63389,#63390,#63391,#63392,#63393,#63394,
#63395,#63396,#63397,#63398,#63399,#63400,#63401,#63402,#63403,#63404,#63405,
#63406,#63407,#63408,#63409,#63410,#63411,#63412,#63413,#63414,#63415,#63416,
#63417,#63418,#63419,#63420,#63421,#63422,#63423,#63424,#63425,#63426,#63427,
#63428,#63429,#63430,#63431,#63432,#63433,#63434,#63435,#63436,#63437,#63438,
#63439,#63440,#63441,#63442,#63443,#63444,#63445,#63446,#63447,#63448,#63449,
#63450,#63451,#63452,#63453,#63454,#63455,#63456,#63457,#63458,#63459,#63460,
#63461,#63462,#63463,#63464,#63465,#63466,#63467,#63468,#63469,#63470,#63471,
#63472),.UNSPECIFIED.,.F.,.F.,(4,3,3,3,3,3,3,3,3,3,3,3,3,3,3,3,3,3,3,3,
3,3,3,3,3,3,3,3,3,3,3,3,3,3,3,3,3,3,3,3,3,3,4),(61.9158792493284,62.0141405915021,
62.1125119987853,62.2109478186409,62.309542353619,62.3427764500624,62.4413745750661,
62.5398323578427,62.6400549256154,62.7383344833436,62.8365810624171,62.9348241454556,
63.0365213340977,63.1349057475165,63.2382593237704,63.3416129000243,63.440211025028,
63.5386688078045,63.6388913755772,63.7371709333053,63.8354175123787,63.9336605954171,
64.0353577840594,64.1337421974782,64.2370957737322,64.3404493499862,64.4390474749898,
64.5375052577665,64.6377278255392,64.7360073832672,64.8342539623407,64.9324970453793,
65.0341942340215,65.1325786474403,65.2359322236942,65.3392857999481,65.4384637976084,
65.5374980774502,65.6364173808603,65.7352455972603,65.8340208922133,65.9327849002203,
65.9734457253857),.UNSPECIFIED.);
#679=B_SPLINE_CURVE_WITH_KNOTS('',3,(#63478,#63479,#63480,#63481,#63482,
#63483,#63484,#63485,#63486,#63487,#63488,#63489,#63490,#63491,#63492,#63493,
#63494,#63495,#63496,#63497,#63498,#63499,#63500,#63501,#63502,#63503,#63504,
#63505,#63506,#63507,#63508,#63509,#63510,#63511,#63512,#63513,#63514,#63515,
#63516,#63517,#63518,#63519,#63520,#63521,#63522,#63523,#63524,#63525,#63526,
#63527,#63528,#63529,#63530,#63531,#63532,#63533,#63534,#63535,#63536,#63537,
#63538,#63539,#63540,#63541,#63542,#63543,#63544,#63545,#63546,#63547,#63548,
#63549,#63550,#63551,#63552,#63553,#63554,#63555,#63556,#63557,#63558,#63559,
#63560,#63561,#63562,#63563,#63564,#63565,#63566,#63567,#63568,#63569,#63570,
#63571,#63572,#63573,#63574,#63575,#63576,#63577,#63578,#63579,#63580,#63581,
#63582,#63583,#63584,#63585,#63586,#63587,#63588,#63589,#63590,#63591,#63592,
#63593,#63594,#63595,#63596,#63597,#63598,#63599,#63600,#63601),
 .UNSPECIFIED.,.F.,.F.,(4,3,3,3,3,3,3,3,3,3,3,3,3,3,3,3,3,3,3,3,3,3,3,3,
3,3,3,3,3,3,3,3,3,3,3,3,3,3,3,3,3,4),(55.6323251840425,55.7308982483116,
55.8157280328489,55.9143261578526,56.0127839406294,56.1130065084021,56.2112860661302,
56.3095326452036,56.4077757282421,56.5094729168843,56.6078573303031,56.7112109065569,
56.8145644828108,56.9131626078145,57.0116203905912,57.1118429583639,57.2101225160921,
57.3083690951655,57.406612178204,57.5083093668461,57.606693780265,57.7100473565188,
57.8134009327727,57.9119990577764,58.010456840553,58.1106794083257,58.2089589660538,
58.3072055451272,58.4054486281657,58.5071458168079,58.6055302302267,58.7088838064806,
58.8122373827345,58.9094791608007,59.0070768179764,59.1040671063403,59.2009981633323,
59.2979009849174,59.3959908432396,59.4929780422902,59.5916192302482,59.6902604182062),
 .UNSPECIFIED.);
#680=B_SPLINE_CURVE_WITH_KNOTS('',3,(#63602,#63603,#63604,#63605,#63606,
#63607,#63608),.UNSPECIFIED.,.F.,.F.,(4,1,1,1,4),(59.6902604182062,59.8110738326964,
60.8099102826583,61.8087467326202,61.9167164720863),.UNSPECIFIED.);
#681=B_SPLINE_CURVE_WITH_KNOTS('',3,(#63610,#63611,#63612,#63613,#63614,
#63615,#63616,#63617,#63618,#63619,#63620,#63621,#63622,#63623,#63624,#63625,
#63626,#63627,#63628,#63629,#63630,#63631,#63632,#63633,#63634,#63635,#63636,
#63637,#63638,#63639,#63640,#63641,#63642,#63643,#63644,#63645,#63646,#63647,
#63648,#63649,#63650,#63651,#63652,#63653,#63654,#63655,#63656,#63657,#63658,
#63659,#63660,#63661,#63662,#63663,#63664,#63665,#63666,#63667,#63668,#63669,
#63670,#63671,#63672,#63673,#63674,#63675,#63676,#63677,#63678,#63679),
 .UNSPECIFIED.,.F.,.F.,(4,3,3,3,3,3,3,3,3,3,3,3,3,3,3,3,3,3,3,3,3,3,3,4),
(59.6902604182062,59.788634173056,59.8869985815969,59.9853827919993,60.0838846667642,
60.1824499292134,60.2811933482972,60.3451035501387,60.4437016751424,60.5421594579191,
60.6423820256918,60.7406615834199,60.8389081624934,60.937151245532,61.0388484341741,
61.1372328475929,61.2405864238468,61.3439400001006,61.4425291322775,61.5409847704297,
61.6393272818776,61.7376024228545,61.835858921854,61.9158792493284),
 .UNSPECIFIED.);
#682=B_SPLINE_CURVE_WITH_KNOTS('',3,(#63680,#63681,#63682,#63683,#63684,
#63685,#63686,#63687,#63688,#63689,#63690,#63691,#63692,#63693,#63694,#63695,
#63696,#63697,#63698,#63699,#63700,#63701,#63702,#63703,#63704,#63705,#63706,
#63707,#63708,#63709,#63710,#63711,#63712,#63713,#63714,#63715,#63716,#63717,
#63718,#63719,#63720,#63721,#63722,#63723,#63724,#63725,#63726,#63727,#63728,
#63729,#63730,#63731,#63732,#63733,#63734,#63735,#63736,#63737,#63738,#63739,
#63740,#63741,#63742,#63743,#63744,#63745,#63746,#63747,#63748,#63749,#63750,
#63751,#63752,#63753,#63754,#63755,#63756,#63757,#63758,#63759,#63760,#63761,
#63762,#63763,#63764,#63765,#63766,#63767,#63768,#63769,#63770,#63771,#63772,
#63773,#63774,#63775,#63776,#63777,#63778,#63779,#63780,#63781,#63782,#63783,
#63784,#63785,#63786,#63787,#63788,#63789,#63790,#63791,#63792,#63793,#63794,
#63795,#63796,#63797,#63798,#63799,#63800,#63801,#63802,#63803),
 .UNSPECIFIED.,.F.,.F.,(4,3,3,3,3,3,3,3,3,3,3,3,3,3,3,3,3,3,3,3,3,3,3,3,
3,3,3,3,3,3,3,3,3,3,3,3,3,3,3,3,3,4),(55.6334625298916,55.7317495743948,
55.8299992179396,55.9282409473069,56.0265042327944,56.12487847957,56.2233185899107,
56.3219158848567,56.3497577502912,56.4483558752948,56.5468136580713,56.6470362258441,
56.7453157835722,56.8435623626454,56.941805445684,57.0435026343263,57.1418870477452,
57.2452406239991,57.3485942002531,57.4471923252568,57.5456501080334,57.6458726758061,
57.7441522335343,57.8423988126077,57.9406418956461,58.0423390842883,58.1407234977071,
58.244077073961,58.3474306502149,58.4460287752186,58.5444865579954,58.644709125768,
58.7429886834962,58.8412352625695,58.939478345608,59.0411755342502,59.1395599476691,
59.242913523923,59.3462671001768,59.4608829140306,59.5755716660049,59.6902604179793),
 .UNSPECIFIED.);
#683=B_SPLINE_CURVE_WITH_KNOTS('',3,(#63809,#63810,#63811,#63812,#63813,
#63814,#63815,#63816),.UNSPECIFIED.,.F.,.F.,(4,1,1,1,1,4),(49.3495871775425,
49.8227093330777,50.8215457830395,51.8203822330014,52.8192186829633,53.4070751110266),
 .UNSPECIFIED.);
#684=B_SPLINE_CURVE_WITH_KNOTS('',3,(#63817,#63818,#63819,#63820,#63821,
#63822,#63823,#63824,#63825,#63826,#63827,#63828,#63829,#63830,#63831,#63832,
#63833,#63834,#63835,#63836,#63837,#63838,#63839,#63840,#63841,#63842,#63843,
#63844,#63845,#63846,#63847,#63848,#63849,#63850,#63851,#63852,#63853,#63854,
#63855,#63856,#63857,#63858,#63859,#63860,#63861,#63862,#63863,#63864,#63865,
#63866,#63867,#63868,#63869,#63870,#63871,#63872,#63873,#63874,#63875,#63876,
#63877,#63878,#63879,#63880,#63881,#63882,#63883,#63884,#63885,#63886),
 .UNSPECIFIED.,.F.,.F.,(4,3,3,3,3,3,3,3,3,3,3,3,3,3,3,3,3,3,3,3,3,3,3,4),
(53.4070755243615,53.5149520672712,53.6231638610662,53.7318758460164,53.8180551329252,
53.9166532579289,54.0151110407057,54.1153336084784,54.2136131662065,54.3118597452799,
54.4101028283183,54.5118000169605,54.6101844303793,54.7135380066332,54.816891582887,
54.9188207830314,55.0172568602171,55.1155965155782,55.2138693470808,55.3121048809365,
55.410364322371,55.5086391351003,55.6069975873545,55.6323251840425),
 .UNSPECIFIED.);
#685=B_SPLINE_CURVE_WITH_KNOTS('',3,(#63888,#63889,#63890,#63891,#63892,
#63893,#63894,#63895,#63896,#63897,#63898,#63899,#63900,#63901,#63902,#63903,
#63904,#63905,#63906,#63907,#63908,#63909,#63910,#63911,#63912,#63913,#63914,
#63915,#63916,#63917,#63918,#63919,#63920,#63921,#63922,#63923,#63924,#63925,
#63926,#63927,#63928,#63929,#63930,#63931,#63932,#63933,#63934,#63935,#63936,
#63937,#63938,#63939,#63940,#63941,#63942,#63943,#63944,#63945,#63946,#63947,
#63948,#63949,#63950,#63951,#63952,#63953,#63954,#63955,#63956,#63957),
 .UNSPECIFIED.,.F.,.F.,(4,3,3,3,3,3,3,3,3,3,3,3,3,3,3,3,3,3,3,3,3,3,3,4),
(53.4070751110266,53.5048543854907,53.6024983707769,53.7000367768843,53.7975186210124,
53.8949743677959,53.9924344477701,54.0899931990353,54.1876041339863,54.2853815723758,
54.3520848503674,54.4506829753712,54.549140758148,54.6493633259206,54.7476428836488,
54.8458894627222,54.9441325457609,55.045829734403,55.1442141478217,55.2475677240755,
55.3509213003293,55.4495112354575,55.5479503969195,55.6334625298916),
 .UNSPECIFIED.);
#686=B_SPLINE_CURVE_WITH_KNOTS('',3,(#63958,#63959,#63960,#63961,#63962,
#63963,#63964,#63965,#63966),.UNSPECIFIED.,.F.,.F.,(4,1,1,1,1,1,4),(49.3496770994594,
49.3579026005581,50.3567390505199,51.3555755004818,52.3544119504437,53.3532484004056,
53.4070751110266),.UNSPECIFIED.);
#687=B_SPLINE_CURVE_WITH_KNOTS('',3,(#63972,#63973,#63974,#63975,#63976,
#63977,#63978,#63979,#63980,#63981,#63982,#63983,#63984,#63985,#63986,#63987,
#63988,#63989,#63990,#63991,#63992,#63993,#63994,#63995,#63996,#63997,#63998,
#63999,#64000,#64001,#64002,#64003,#64004,#64005,#64006,#64007,#64008,#64009,
#64010,#64011,#64012,#64013,#64014,#64015,#64016,#64017,#64018,#64019,#64020,
#64021,#64022,#64023,#64024,#64025,#64026,#64027,#64028,#64029,#64030,#64031,
#64032,#64033,#64034,#64035,#64036,#64037,#64038,#64039,#64040,#64041,#64042,
#64043,#64044,#64045,#64046,#64047,#64048,#64049,#64050,#64051,#64052,#64053,
#64054,#64055,#64056,#64057,#64058,#64059,#64060,#64061,#64062,#64063,#64064,
#64065,#64066,#64067,#64068,#64069,#64070,#64071,#64072,#64073,#64074,#64075,
#64076,#64077,#64078,#64079,#64080,#64081,#64082,#64083,#64084,#64085,#64086,
#64087,#64088,#64089,#64090,#64091,#64092,#64093,#64094,#64095),
 .UNSPECIFIED.,.F.,.F.,(4,3,3,3,3,3,3,3,3,3,3,3,3,3,3,3,3,3,3,3,3,3,3,3,
3,3,3,3,3,3,3,3,3,3,3,3,3,3,3,3,3,4),(43.0671358249316,43.1654506744533,
43.2637142379643,43.3619560191833,43.4602054928574,43.558557934537,43.6569637792126,
43.7555405534103,43.8296906333064,43.9282887583115,44.0267465410897,44.126969108862,
44.2252486665916,44.3234952456663,44.4217383287061,44.5234355173466,44.6218199307669,
44.7251735070176,44.8285270832683,44.9271252082716,45.0255829910478,45.1258055588206,
45.2240851165483,45.3223316956211,45.4205747786593,45.5222719673021,45.6206563807204,
45.7240099569753,45.8273635332302,45.9259616582338,46.0244194410105,46.1246420087832,
46.2229215665111,46.3211681455844,46.4194112286225,46.5211084172649,46.6194928306835,
46.7228464069377,46.826199983192,46.9466622822341,47.0654828012636,47.1238896269672),
 .UNSPECIFIED.);
#688=B_SPLINE_CURVE_WITH_KNOTS('',3,(#64096,#64097,#64098,#64099,#64100,
#64101),.UNSPECIFIED.,.F.,.F.,(4,1,1,4),(47.123889803847,47.8250364331539,
48.8238728831158,49.3495871775425),.UNSPECIFIED.);
#689=B_SPLINE_CURVE_WITH_KNOTS('',3,(#64103,#64104,#64105,#64106,#64107,
#64108),.UNSPECIFIED.,.F.,.F.,(4,1,1,4),(47.1238901033263,47.3602297006343,
48.3590661505962,49.3496770994594),.UNSPECIFIED.);
#690=B_SPLINE_CURVE_WITH_KNOTS('',3,(#64109,#64110,#64111,#64112,#64113,
#64114,#64115,#64116,#64117,#64118,#64119,#64120,#64121,#64122,#64123,#64124,
#64125,#64126,#64127,#64128,#64129,#64130,#64131,#64132,#64133,#64134,#64135,
#64136,#64137,#64138,#64139,#64140,#64141,#64142,#64143,#64144,#64145,#64146,
#64147,#64148,#64149,#64150,#64151,#64152,#64153,#64154,#64155,#64156,#64157,
#64158,#64159,#64160,#64161,#64162,#64163,#64164,#64165,#64166,#64167,#64168,
#64169,#64170,#64171,#64172,#64173,#64174,#64175,#64176,#64177,#64178,#64179,
#64180,#64181,#64182,#64183,#64184,#64185,#64186,#64187,#64188,#64189,#64190,
#64191,#64192,#64193,#64194,#64195,#64196,#64197,#64198,#64199,#64200,#64201,
#64202,#64203,#64204,#64205,#64206,#64207,#64208,#64209,#64210,#64211,#64212,
#64213,#64214,#64215,#64216,#64217,#64218,#64219,#64220,#64221,#64222,#64223,
#64224,#64225,#64226,#64227,#64228,#64229,#64230,#64231,#64232),
 .UNSPECIFIED.,.F.,.F.,(4,3,3,3,3,3,3,3,3,3,3,3,3,3,3,3,3,3,3,3,3,3,3,3,
3,3,3,3,3,3,3,3,3,3,3,3,3,3,3,3,3,4),(43.0660207696421,43.1644088774625,
43.2646463891246,43.3648839007868,43.4634820258003,43.5619398085869,43.6621623763571,
43.7604419340954,43.858688513179,43.956931596228,44.0586287848581,44.1570131982874,
44.260366774518,44.3637203507487,44.4623184757497,44.5607762585235,44.6609988262969,
44.7592783840224,44.8575249630931,44.9557680461289,45.0574652347743,45.1558496481904,
45.2592032244505,45.3625568007106,45.4611549257132,45.5596127084888,45.6598352762618,
45.7581148339887,45.856361413061,45.9546044960978,46.0563016847414,46.1546860981589,
46.2580396744157,46.3613932506724,46.4587199838046,46.5559210250952,46.6530274701203,
46.7500702965179,46.8471124553621,46.9441490048064,47.0412721236584,47.123889803847),
 .UNSPECIFIED.);
#691=B_SPLINE_CURVE_WITH_KNOTS('',3,(#64238,#64239,#64240,#64241,#64242,
#64243,#64244,#64245,#64246,#64247,#64248,#64249,#64250,#64251,#64252,#64253,
#64254,#64255,#64256,#64257,#64258,#64259,#64260,#64261,#64262,#64263,#64264,
#64265,#64266,#64267,#64268,#64269,#64270,#64271,#64272,#64273,#64274,#64275,
#64276,#64277,#64278,#64279,#64280,#64281,#64282,#64283,#64284,#64285,#64286,
#64287,#64288,#64289,#64290,#64291,#64292,#64293,#64294,#64295,#64296,#64297,
#64298,#64299,#64300,#64301,#64302,#64303,#64304,#64305,#64306,#64307,#64308,
#64309,#64310,#64311,#64312,#64313,#64314,#64315,#64316,#64317,#64318,#64319,
#64320,#64321,#64322,#64323,#64324,#64325,#64326,#64327,#64328,#64329,#64330,
#64331,#64332,#64333,#64334,#64335,#64336,#64337,#64338,#64339,#64340,#64341,
#64342,#64343,#64344,#64345,#64346,#64347,#64348,#64349,#64350,#64351,#64352,
#64353,#64354,#64355,#64356,#64357,#64358,#64359,#64360,#64361,#64362,#64363,
#64364),.UNSPECIFIED.,.F.,.F.,(4,3,3,3,3,3,3,3,3,3,3,3,3,3,3,3,3,3,3,3,
3,3,3,3,3,3,3,3,3,3,3,3,3,3,3,3,3,3,3,3,3,3,4),(36.7830721123744,36.8378354835733,
36.9364336084867,37.0348913911713,37.1351139589668,37.2333935165991,37.3316400955754,
37.4298831785158,37.5315803672706,37.6299647805896,37.7333183570624,37.8366719335352,
37.9352700586076,38.0337278414541,38.1339504092095,38.2322299670092,38.3304765461547,
38.4287196292657,38.5304168178235,38.6288012313153,38.7321548074061,38.835508383497,
38.9341065084864,39.0325642912488,39.132786859025,39.2310664167388,39.3293129957978,
39.4275560788219,39.5292532674812,39.6276376808859,39.7309912571724,39.8343448334589,
39.9329429584521,40.0314007412181,40.1316233089934,40.2299028667104,40.3281494457725,
40.4263925287995,40.5280897174548,40.6264741308619,40.7298277071414,40.8331812834208,
40.8407044966674),.UNSPECIFIED.);
#692=B_SPLINE_CURVE_WITH_KNOTS('',3,(#64365,#64366,#64367,#64368,#64369,
#64370,#64371,#64372,#64373,#64374,#64375,#64376,#64377,#64378,#64379,#64380,
#64381,#64382,#64383,#64384,#64385,#64386,#64387,#64388,#64389,#64390,#64391,
#64392,#64393,#64394,#64395,#64396,#64397,#64398,#64399,#64400,#64401,#64402,
#64403,#64404,#64405,#64406,#64407,#64408,#64409,#64410,#64411,#64412,#64413,
#64414,#64415,#64416,#64417,#64418,#64419,#64420,#64421,#64422,#64423,#64424,
#64425,#64426,#64427,#64428,#64429,#64430,#64431,#64432,#64433,#64434),
 .UNSPECIFIED.,.F.,.F.,(4,3,3,3,3,3,3,3,3,3,3,3,3,3,3,3,3,3,3,3,3,3,3,4),
(40.8407044969197,40.9391705387198,41.037496428004,41.1368115911763,41.2349607512892,
41.3330774110127,41.4311912274061,41.5313978539003,41.6296531901072,41.730835461745,
41.8320177333827,41.9306158583838,42.029073641158,42.1292962089313,42.2275757666567,
42.3258223457274,42.4240654287631,42.5257626174084,42.6241470308246,42.7275006070845,
42.8308541833445,42.9294559188181,43.0279051778381,43.0671358249316),
 .UNSPECIFIED.);
#693=B_SPLINE_CURVE_WITH_KNOTS('',3,(#64436,#64437,#64438,#64439,#64440,
#64441,#64442,#64443,#64444,#64445,#64446,#64447,#64448,#64449,#64450,#64451,
#64452,#64453,#64454,#64455,#64456,#64457,#64458,#64459,#64460,#64461,#64462,
#64463,#64464,#64465,#64466,#64467,#64468,#64469,#64470,#64471,#64472,#64473,
#64474,#64475,#64476,#64477,#64478,#64479,#64480,#64481,#64482,#64483,#64484,
#64485,#64486,#64487,#64488,#64489,#64490,#64491,#64492,#64493,#64494,#64495,
#64496,#64497,#64498,#64499,#64500,#64501,#64502,#64503,#64504,#64505),
 .UNSPECIFIED.,.F.,.F.,(4,3,3,3,3,3,3,3,3,3,3,3,3,3,3,3,3,3,3,3,3,3,3,4),
(40.8407044966674,40.9425310419933,41.0487010317108,41.1508691915798,41.2531658485548,
41.3556785603237,41.3672110008631,41.4658091258525,41.5642669086149,41.6644894763912,
41.7627690341049,41.8610156131639,41.959258696188,42.0609558848472,42.159340298252,
42.2626938745384,42.3660474508249,42.4646234053317,42.5630692109038,42.6614145832016,
42.7625661298117,42.8608128923214,42.9634168309817,43.0660207696421),
 .UNSPECIFIED.);
#694=B_SPLINE_CURVE_WITH_KNOTS('',3,(#64506,#64507,#64508,#64509,#64510,
#64511,#64512,#64513),.UNSPECIFIED.,.F.,.F.,(4,1,1,1,1,4),(36.7838197774947,
37.3718652010156,38.3707016509774,39.3695381009393,40.3683745509012,40.8407024148877),
 .UNSPECIFIED.);
#695=B_SPLINE_CURVE_WITH_KNOTS('',3,(#64519,#64520,#64521,#64522,#64523,
#64524,#64525,#64526,#64527,#64528,#64529,#64530,#64531,#64532,#64533,#64534,
#64535,#64536,#64537,#64538,#64539,#64540,#64541,#64542,#64543,#64544,#64545,
#64546,#64547,#64548,#64549,#64550,#64551,#64552,#64553,#64554,#64555,#64556,
#64557,#64558,#64559,#64560,#64561,#64562,#64563,#64564,#64565,#64566,#64567,
#64568,#64569,#64570,#64571,#64572,#64573,#64574,#64575,#64576,#64577,#64578,
#64579,#64580,#64581,#64582,#64583,#64584,#64585,#64586,#64587,#64588,#64589,
#64590,#64591,#64592,#64593,#64594,#64595,#64596,#64597,#64598,#64599,#64600,
#64601,#64602,#64603,#64604,#64605,#64606,#64607,#64608,#64609,#64610,#64611,
#64612,#64613,#64614,#64615,#64616,#64617,#64618,#64619,#64620,#64621,#64622,
#64623,#64624,#64625,#64626,#64627,#64628,#64629,#64630,#64631,#64632,#64633,
#64634,#64635,#64636,#64637,#64638,#64639,#64640,#64641,#64642,#64643,#64644,
#64645),.UNSPECIFIED.,.F.,.F.,(4,3,3,3,3,3,3,3,3,3,3,3,3,3,3,3,3,3,3,3,
3,3,3,3,3,3,3,3,3,3,3,3,3,3,3,3,3,3,3,3,3,3,4),(30.4997391997366,30.5981024250019,
30.6965256310033,30.7951123412346,30.844816783802,30.9434149029217,31.0418726797114,
31.1420952489679,31.240374800498,31.3386213733081,31.4368644500261,31.5385616459606,
31.6369460529803,31.7402996433721,31.8436532337639,31.9422513619701,32.0407091479896,
32.1409317149566,32.2392112760025,32.3374578584144,32.4357009448076,32.5373981295371,
32.6357825463172,32.7391361150215,32.8424896837258,32.941087808515,33.0395455910825,
33.1397681589082,33.2380477164417,33.3362942953263,33.4345373781827,33.5362345670589,
33.6346189803128,33.7379725570002,33.8413261336877,33.9390973941506,34.0367388270547,
34.1342810926888,34.2317547370042,34.3292101035739,34.4266554953284,34.5241539309046,
34.5575191894878),.UNSPECIFIED.);
#696=B_SPLINE_CURVE_WITH_KNOTS('',3,(#64646,#64647,#64648,#64649,#64650,
#64651,#64652,#64653,#64654,#64655,#64656,#64657,#64658,#64659,#64660,#64661,
#64662,#64663,#64664,#64665,#64666,#64667,#64668,#64669,#64670,#64671,#64672,
#64673,#64674,#64675,#64676,#64677,#64678,#64679,#64680,#64681,#64682,#64683,
#64684,#64685,#64686,#64687,#64688,#64689,#64690,#64691,#64692,#64693,#64694,
#64695,#64696,#64697,#64698,#64699,#64700,#64701,#64702,#64703,#64704,#64705,
#64706,#64707,#64708,#64709,#64710,#64711,#64712,#64713,#64714,#64715),
 .UNSPECIFIED.,.F.,.F.,(4,3,3,3,3,3,3,3,3,3,3,3,3,3,3,3,3,3,3,3,3,3,3,4),
(34.5575191897594,34.6782345503652,34.8009387396128,34.8401625836495,34.938760709128,
35.0372184923859,35.1374410600391,35.2357206182603,35.3339671978303,35.4322102813681,
35.5339074694289,35.6322918833488,35.7356454584801,35.8389990336114,35.9376008413523,
36.0360613066058,36.1344037647061,36.2326817408451,36.3309247589454,36.4291623016109,
36.5274785677124,36.625837103631,36.724338350044,36.7830721123744),
 .UNSPECIFIED.);
#697=B_SPLINE_CURVE_WITH_KNOTS('',3,(#64717,#64718,#64719,#64720,#64721,
#64722),.UNSPECIFIED.,.F.,.F.,(4,1,1,4),(34.5575241466493,35.3741923010918,
36.3730287510537,36.7838197774947),.UNSPECIFIED.);
#698=B_SPLINE_CURVE_WITH_KNOTS('',3,(#64723,#64724,#64725,#64726,#64727,
#64728,#64729,#64730,#64731,#64732,#64733,#64734,#64735,#64736,#64737,#64738,
#64739,#64740,#64741,#64742,#64743,#64744,#64745,#64746,#64747,#64748,#64749,
#64750,#64751,#64752,#64753,#64754,#64755,#64756,#64757,#64758,#64759,#64760,
#64761,#64762,#64763,#64764,#64765,#64766,#64767,#64768,#64769,#64770,#64771,
#64772,#64773,#64774,#64775,#64776,#64777,#64778,#64779,#64780,#64781,#64782,
#64783,#64784,#64785,#64786,#64787,#64788,#64789,#64790,#64791,#64792,#64793,
#64794,#64795,#64796,#64797,#64798,#64799,#64800,#64801,#64802,#64803,#64804,
#64805,#64806,#64807,#64808,#64809,#64810,#64811,#64812,#64813,#64814,#64815,
#64816,#64817,#64818,#64819,#64820,#64821,#64822,#64823,#64824,#64825,#64826,
#64827,#64828,#64829,#64830,#64831,#64832,#64833,#64834,#64835,#64836,#64837,
#64838,#64839,#64840,#64841,#64842,#64843,#64844,#64845,#64846),
 .UNSPECIFIED.,.F.,.F.,(4,3,3,3,3,3,3,3,3,3,3,3,3,3,3,3,3,3,3,3,3,3,3,3,
3,3,3,3,3,3,3,3,3,3,3,3,3,3,3,3,3,4),(30.5006744364989,30.5991052402592,
30.6974320357731,30.7957023845,30.8939457980153,30.9921917542775,31.0905375391577,
31.1889321006504,31.2875030416228,31.3788465012443,31.4774446473005,31.575902451375,
31.6761250138539,31.7744045933259,31.8726511942622,31.9708942992537,32.0725914622418,
32.1709758976143,32.2743294244103,32.3776829512062,32.4762810765929,32.5747388598192,
32.6749614274878,32.7732409858268,32.8714875655702,32.9697306493373,33.071427837295,
33.169812251582,33.2731658263751,33.3765194011681,33.4751175202855,33.5735752970726,
33.6737978663298,33.7720774178574,33.8703239906649,33.9685670673804,34.0702642633178,
34.1686486703349,34.2720022607324,34.37535585113,34.5238559810743,34.5575191894878),
 .UNSPECIFIED.);
#699=B_SPLINE_CURVE_WITH_KNOTS('',3,(#64852,#64853,#64854,#64855,#64856,
#64857,#64858,#64859),.UNSPECIFIED.,.F.,.F.,(4,1,1,1,1,4),(24.2176478004184,
24.8517980840308,25.8506345339927,26.8494709839545,27.8483074339164,28.2743284148783),
 .UNSPECIFIED.);
#700=B_SPLINE_CURVE_WITH_KNOTS('',3,(#64860,#64861,#64862,#64863,#64864,
#64865,#64866,#64867,#64868,#64869,#64870,#64871,#64872,#64873,#64874,#64875,
#64876,#64877,#64878,#64879,#64880,#64881,#64882,#64883,#64884,#64885,#64886,
#64887,#64888,#64889,#64890,#64891,#64892,#64893,#64894,#64895,#64896,#64897,
#64898,#64899,#64900,#64901,#64902,#64903,#64904,#64905,#64906,#64907,#64908,
#64909,#64910,#64911,#64912,#64913,#64914,#64915,#64916,#64917,#64918,#64919,
#64920,#64921,#64922,#64923,#64924,#64925,#64926,#64927,#64928,#64929),
 .UNSPECIFIED.,.F.,.F.,(4,3,3,3,3,3,3,3,3,3,3,3,3,3,3,3,3,3,3,3,3,3,3,4),
(28.2743338823082,28.3746245107026,28.4749734040128,28.5754886322331,28.6760922705589,
28.7769068627545,28.8471438838783,28.9457420299255,29.0441998339908,29.144422396472,
29.2427019759346,29.3409485768615,29.4391916818436,29.5408888448427,29.6392732802058,
29.742626807023,29.8459803338402,29.9445606477241,30.0430096057709,30.1413569295411,
30.2396381186526,30.3378792535374,30.4361386871576,30.4997391997366),
 .UNSPECIFIED.);
#701=B_SPLINE_CURVE_WITH_KNOTS('',3,(#64931,#64932,#64933,#64934,#64935,
#64936,#64937,#64938,#64939,#64940,#64941,#64942,#64943,#64944,#64945,#64946,
#64947,#64948,#64949,#64950,#64951,#64952,#64953,#64954,#64955,#64956,#64957,
#64958,#64959,#64960,#64961,#64962,#64963,#64964,#64965,#64966,#64967,#64968,
#64969,#64970,#64971,#64972,#64973,#64974,#64975,#64976,#64977,#64978,#64979,
#64980,#64981,#64982,#64983,#64984,#64985,#64986,#64987,#64988,#64989,#64990,
#64991,#64992,#64993,#64994,#64995,#64996,#64997,#64998,#64999,#65000),
 .UNSPECIFIED.,.F.,.F.,(4,3,3,3,3,3,3,3,3,3,3,3,3,3,3,3,3,3,3,3,3,3,3,4),
(28.2743338823082,28.3823371513587,28.4809354104368,28.5793933287022,28.6796158627795,
28.7778955584748,28.8761422761379,28.9743854982056,29.0760825239843,29.1744670761058,
29.2778203387132,29.3811736013206,29.4797717427275,29.5782295425788,29.6784521061668,
29.7767316825037,29.8749782807199,29.9732213834117,30.0749185503794,30.1733029845339,
30.2766565179082,30.3800100512825,30.4786103665625,30.5006744364989),
 .UNSPECIFIED.);
#702=B_SPLINE_CURVE_WITH_KNOTS('',3,(#65001,#65002,#65003,#65004,#65005,
#65006,#65007,#65008,#65009,#65010,#65011,#65012,#65013,#65014,#65015,#65016,
#65017,#65018,#65019,#65020,#65021,#65022,#65023,#65024,#65025,#65026,#65027,
#65028,#65029,#65030,#65031,#65032,#65033,#65034,#65035,#65036,#65037,#65038,
#65039,#65040,#65041,#65042,#65043,#65044,#65045,#65046,#65047,#65048,#65049,
#65050,#65051,#65052,#65053,#65054,#65055,#65056,#65057,#65058,#65059,#65060,
#65061,#65062,#65063,#65064,#65065,#65066,#65067,#65068,#65069,#65070,#65071,
#65072,#65073,#65074,#65075,#65076,#65077,#65078,#65079,#65080,#65081,#65082,
#65083,#65084,#65085,#65086,#65087,#65088,#65089,#65090,#65091,#65092,#65093,
#65094,#65095,#65096,#65097,#65098,#65099,#65100,#65101,#65102,#65103,#65104,
#65105,#65106,#65107,#65108,#65109,#65110,#65111,#65112,#65113,#65114,#65115,
#65116,#65117,#65118,#65119,#65120,#65121,#65122,#65123,#65124,#65125,#65126,
#65127),.UNSPECIFIED.,.F.,.F.,(4,3,3,3,3,3,3,3,3,3,3,3,3,3,3,3,3,3,3,3,
3,3,3,3,3,3,3,3,3,3,3,3,3,3,3,3,3,3,3,3,3,3,4),(24.2164091062169,24.3149891554594,
24.3869913515112,24.4855869755136,24.5840422190559,24.6842654168581,24.7825423598393,
24.8807863016633,24.9790267283841,25.0807269966564,25.1791087331383,25.2824682673057,
25.3858278014731,25.4844267472597,25.5828853582973,25.6831077199395,25.7813881181849,
25.8796355405022,25.9778794683927,26.0795756641532,26.1779609177654,26.2813125846002,
26.384664251435,26.4832625890263,26.5817205904922,26.6819431043553,26.7802228942346,
26.8784697099906,26.976713033946,27.0784099508087,27.1767946133168,27.2801476573568,
27.3835007013968,27.4808124349029,27.5800026158,27.6770619108145,27.7740624128206,
27.8710350559302,27.9718597624675,28.0689211605358,28.1660361013683,28.2632831488084,
28.2743338820795),.UNSPECIFIED.);
#703=B_SPLINE_CURVE_WITH_KNOTS('',3,(#65133,#65134,#65135,#65136,#65137,
#65138),.UNSPECIFIED.,.F.,.F.,(4,1,1,4),(15.707963267949,16.3962997518162,
17.3951362017781,17.9335273147171),.UNSPECIFIED.);
#704=B_SPLINE_CURVE_WITH_KNOTS('',3,(#65140,#65141,#65142,#65143,#65144),
 .UNSPECIFIED.,.F.,.F.,(4,1,4),(14.3986268518925,15.3974633018543,15.707963267949),
 .UNSPECIFIED.);
#705=B_SPLINE_CURVE_WITH_KNOTS('',3,(#65148,#65149,#65150,#65151,#65152,
#65153,#65154,#65155,#65156,#65157,#65158,#65159,#65160,#65161,#65162,#65163,
#65164,#65165,#65166,#65167,#65168,#65169,#65170,#65171,#65172,#65173,#65174,
#65175,#65176,#65177,#65178,#65179,#65180,#65181,#65182,#65183,#65184,#65185,
#65186,#65187,#65188,#65189,#65190,#65191,#65192,#65193,#65194,#65195,#65196,
#65197,#65198,#65199,#65200,#65201,#65202,#65203,#65204,#65205),
 .UNSPECIFIED.,.F.,.F.,(4,3,3,3,3,3,3,3,3,3,3,3,3,3,3,3,3,3,3,4),(13.8757070305535,
13.9742334885845,14.0726196430263,14.1714713856995,14.2696800147308,14.3678555358063,
14.4660275256487,14.5653790403395,14.6636889428954,14.7635612636537,14.8634335844121,
14.9606976643214,15.0578044061946,15.154822904629,15.2517842090804,15.3487192963901,
15.4457083601634,15.5427241599105,15.6398692512359,15.707963267949),
 .UNSPECIFIED.);
#706=B_SPLINE_CURVE_WITH_KNOTS('',3,(#65206,#65207,#65208,#65209,#65210,
#65211,#65212),.UNSPECIFIED.,.F.,.F.,(4,1,1,1,4),(15.707963267949,15.8622700343739,
16.8611064843358,17.8599429342977,17.9342415705864),.UNSPECIFIED.);
#707=B_SPLINE_CURVE_WITH_KNOTS('',3,(#65218,#65219,#65220,#65221,#65222,
#65223,#65224,#65225,#65226,#65227,#65228,#65229,#65230,#65231,#65232,#65233,
#65234,#65235,#65236,#65237,#65238,#65239,#65240,#65241,#65242,#65243,#65244,
#65245,#65246,#65247,#65248,#65249,#65250,#65251,#65252,#65253,#65254,#65255),
 .UNSPECIFIED.,.F.,.F.,(4,2,2,2,2,2,2,2,2,2,2,2,2,2,2,2,2,2,4),(2.08269229218369E-5,
0.127845741022052,0.200677725447424,0.317389539257015,0.404625699897331,
0.484292562096328,0.651098313987348,0.735080070424923,0.809478158094123,
0.977078046750801,1.04711496328757,1.11953227018629,1.23167820677694,1.31165216412917,
1.44942689358888,1.5844225186206,1.6597570912359,1.79045634738967,1.80127748042845),
 .UNSPECIFIED.);
#708=B_SPLINE_CURVE_WITH_KNOTS('',3,(#65259,#65260,#65261,#65262,#65263,
#65264,#65265,#65266,#65267,#65268,#65269,#65270,#65271,#65272,#65273),
 .UNSPECIFIED.,.F.,.F.,(4,1,1,1,1,1,1,1,1,1,1,1,4),(2.02178176728025,2.43673748880502,
2.92408498656602,3.41143248432702,3.89877998208802,4.38612747984902,4.87347497761003,
5.36082247537103,5.84816997313203,6.33551747089303,6.82286496865404,7.31021246641504,
7.59153924858055),.UNSPECIFIED.);
#709=B_SPLINE_CURVE_WITH_KNOTS('',3,(#65274,#65275,#65276,#65277,#65278,
#65279,#65280,#65281,#65282,#65283,#65284,#65285,#65286,#65287,#65288,#65289),
 .UNSPECIFIED.,.F.,.F.,(4,3,3,3,3,4),(7.59153924858055,7.6845224783778,
7.77753299194073,7.79755996417604,7.88865013802183,7.94826257243732),
 .UNSPECIFIED.);
#710=B_SPLINE_CURVE_WITH_KNOTS('',3,(#65295,#65296,#65297,#65298,#65299,
#65300,#65301,#65302,#65303,#65304,#65305,#65306,#65307),.UNSPECIFIED.,
 .F.,.F.,(4,3,3,3,4),(-10.494778244858,-10.4064615792516,-10.3181205168946,
-10.2342974529811,-10.1382057107015),.UNSPECIFIED.);
#711=B_SPLINE_CURVE_WITH_KNOTS('',3,(#65308,#65309,#65310,#65311,#65312,
#65313,#65314,#65315,#65316,#65317,#65318,#65319,#65320,#65321,#65322,#65323,
#65324,#65325,#65326,#65327,#65328,#65329,#65330,#65331,#65332,#65333,#65334,
#65335,#65336,#65337,#65338,#65339,#65340,#65341,#65342,#65343,#65344,#65345,
#65346,#65347,#65348,#65349,#65350,#65351,#65352,#65353,#65354,#65355,#65356,
#65357,#65358,#65359,#65360,#65361),.UNSPECIFIED.,.F.,.F.,(4,2,2,2,2,2,
2,2,2,2,2,2,2,2,2,2,2,2,2,2,2,2,2,2,2,2,4),(1.80127748042845,1.89084368471754,
1.95813908989248,2.04086238183236,2.16780801322339,2.30159594752158,2.38018362026978,
2.50753564499175,2.58026582803546,2.72352856314932,2.80831445209385,2.89229737147604,
3.05890113029296,3.13853522888799,3.22570967551258,3.30970314422656,3.47395562175451,
3.55354130187497,3.69234485228637,3.77242982395912,3.83814226949863,3.88038829310432,
3.95516208872894,4.02096865651561,4.17915166056594,4.2564735047848,4.33558734702027),
 .UNSPECIFIED.);
#712=B_SPLINE_CURVE_WITH_KNOTS('',3,(#65363,#65364,#65365,#65366,#65367,
#65368,#65369,#65370,#65371,#65372,#65373,#65374,#65375,#65376,#65377,#65378,
#65379,#65380,#65381,#65382,#65383,#65384,#65385,#65386,#65387,#65388,#65389,
#65390,#65391,#65392,#65393,#65394,#65395,#65396,#65397,#65398,#65399,#65400,
#65401,#65402,#65403,#65404,#65405,#65406,#65407,#65408,#65409,#65410,#65411,
#65412,#65413,#65414,#65415,#65416,#65417,#65418,#65419,#65420,#65421,#65422,
#65423,#65424,#65425,#65426,#65427,#65428,#65429,#65430,#65431,#65432,#65433,
#65434,#65435,#65436,#65437,#65438,#65439,#65440,#65441,#65442,#65443,#65444,
#65445,#65446,#65447,#65448,#65449,#65450,#65451,#65452,#65453,#65454,#65455,
#65456,#65457,#65458,#65459,#65460,#65461,#65462,#65463,#65464,#65465,#65466,
#65467,#65468,#65469,#65470,#65471,#65472,#65473,#65474,#65475,#65476,#65477,
#65478,#65479,#65480,#65481,#65482,#65483,#65484,#65485,#65486,#65487,#65488,
#65489,#65490,#65491,#65492,#65493,#65494,#65495,#65496,#65497,#65498,#65499,
#65500,#65501,#65502,#65503,#65504,#65505,#65506,#65507,#65508,#65509,#65510,
#65511,#65512,#65513,#65514,#65515,#65516,#65517,#65518,#65519,#65520,#65521,
#65522,#65523,#65524,#65525,#65526,#65527,#65528,#65529,#65530,#65531,#65532,
#65533,#65534,#65535,#65536,#65537,#65538,#65539,#65540,#65541,#65542,#65543,
#65544,#65545,#65546,#65547,#65548,#65549,#65550,#65551,#65552,#65553,#65554,
#65555,#65556,#65557,#65558,#65559,#65560,#65561,#65562,#65563,#65564,#65565,
#65566,#65567,#65568,#65569,#65570,#65571,#65572,#65573),.UNSPECIFIED.,
 .F.,.F.,(4,3,3,3,3,3,3,3,3,3,3,3,3,3,3,3,3,3,3,3,3,3,3,3,3,3,3,3,3,3,3,
3,3,3,3,3,3,3,3,3,3,3,3,3,3,3,3,3,3,3,3,3,3,3,3,3,3,3,3,3,3,3,3,3,3,3,3,
3,3,3,4),(7.94826257243732,8.03933927732266,8.13040900661477,8.22150087575582,
8.28490746193705,8.37600661966196,8.46708750385086,8.55817107950977,8.64925032934137,
8.7403486849684,8.77225495969805,8.86358446014535,8.95489727790249,9.04621272797726,
9.13752315628156,9.22884970421161,9.25960245745905,9.35004563389331,9.44046838421938,
9.53089683726842,9.62132426183796,9.71178086513476,9.74694995522005,9.83977082466953,
9.93258020493847,10.0253815422507,10.1181658427925,10.2109349487687,10.2342974529811,
10.3226340982603,10.4109484628818,10.4992807310775,10.5876214045936,10.6760195929041,
10.7216449507421,10.8172935625052,10.9152182840046,11.0107916985716,11.1098920735374,
11.2089924485031,11.2974475293379,11.3858999834853,11.4743988429813,11.5629222999095,
11.6515265886469,11.6963399462641,11.7845988436236,11.8727845281299,11.96091671564,
12.0496814939083,12.1377836965724,12.2258943659517,12.3140313137176,12.4032822207347,
12.4915724815489,12.5813037116675,12.6710349417861,12.7563666072233,12.8415825207838,
12.9267064287632,13.0117619568872,13.0967819333776,13.1817864079043,13.2667966276969,
13.3518338433476,13.4369714570383,13.5221663247904,13.6074971372277,13.6457299373081,
13.7757706988632,13.8747245557601),.UNSPECIFIED.);
#713=B_SPLINE_CURVE_WITH_KNOTS('',3,(#65574,#65575,#65576,#65577,#65578,
#65579,#65580,#65581,#65582,#65583,#65584,#65585,#65586,#65587,#65588,#65589),
 .UNSPECIFIED.,.F.,.F.,(4,3,3,3,3,4),(13.8747245559393,13.964019218205,
14.0502847363995,14.1364982676294,14.222679165221,14.2319032050023),
 .UNSPECIFIED.);
#714=B_SPLINE_CURVE_WITH_KNOTS('',3,(#65595,#65596,#65597,#65598,#65599,
#65600),.UNSPECIFIED.,.F.,.F.,(4,2,4),(-0.153225104208862,-0.0777958673852031,
-0.000838790028883987),.UNSPECIFIED.);
#715=B_SPLINE_CURVE_WITH_KNOTS('',3,(#65601,#65602,#65603,#65604,#65605,
#65606,#65607,#65608,#65609,#65610,#65611,#65612,#65613,#65614,#65615,#65616,
#65617,#65618,#65619,#65620,#65621,#65622,#65623,#65624,#65625,#65626,#65627,
#65628,#65629,#65630,#65631,#65632,#65633,#65634,#65635,#65636,#65637,#65638,
#65639,#65640,#65641,#65642,#65643,#65644,#65645,#65646,#65647,#65648,#65649,
#65650,#65651,#65652,#65653,#65654,#65655,#65656,#65657,#65658,#65659,#65660,
#65661,#65662,#65663,#65664,#65665,#65666,#65667,#65668,#65669,#65670,#65671,
#65672,#65673,#65674,#65675,#65676,#65677,#65678,#65679,#65680,#65681,#65682,
#65683,#65684,#65685,#65686,#65687,#65688,#65689,#65690,#65691,#65692,#65693,
#65694,#65695,#65696,#65697,#65698,#65699,#65700,#65701,#65702,#65703,#65704,
#65705,#65706,#65707,#65708,#65709,#65710,#65711,#65712,#65713,#65714,#65715,
#65716,#65717,#65718,#65719,#65720,#65721,#65722,#65723,#65724,#65725,#65726,
#65727,#65728,#65729,#65730,#65731,#65732,#65733,#65734,#65735,#65736,#65737,
#65738,#65739,#65740,#65741,#65742,#65743,#65744,#65745,#65746,#65747,#65748,
#65749,#65750,#65751,#65752,#65753,#65754,#65755,#65756,#65757,#65758,#65759,
#65760,#65761,#65762,#65763,#65764,#65765,#65766,#65767,#65768,#65769,#65770,
#65771,#65772,#65773,#65774,#65775,#65776,#65777,#65778,#65779,#65780,#65781,
#65782,#65783,#65784,#65785,#65786,#65787,#65788,#65789,#65790,#65791,#65792,
#65793,#65794,#65795,#65796,#65797,#65798,#65799,#65800,#65801,#65802,#65803,
#65804,#65805,#65806,#65807,#65808),.UNSPECIFIED.,.F.,.F.,(4,3,3,3,3,3,
3,3,3,3,3,3,3,3,3,3,3,3,3,3,3,3,3,3,3,3,3,3,3,3,3,3,3,3,3,3,3,3,3,3,3,3,
3,3,3,3,3,3,3,3,3,3,3,3,3,3,3,3,3,3,3,3,3,3,3,3,3,3,3,4),(-16.4213910178811,
-16.3286432460334,-16.2359126775523,-16.1431937736906,-16.0824674261131,
-15.9941326347525,-15.9058201280992,-15.81748971347,-15.7291508902718,-15.6407545361228,
-15.5951199283521,-15.4994686331016,-15.401544582474,-15.3059685045778,
-15.2068704675844,-15.1077724305911,-15.0193184286812,-14.9308670580831,
-14.8423692825813,-14.7538469094734,-14.6652436972666,-14.6204249328301,
-14.5321659959703,-14.4439802741915,-14.3558480516816,-14.2670832873849,
-14.1789810556079,-14.0908703594027,-14.0027333871464,-13.9134825246869,
-13.8251922454331,-13.7354610913706,-13.6457299373081,-13.5603980691463,
-13.4751819518284,-13.3900578392207,-13.3050021057494,-13.2199819233987,
-13.134977242644,-13.0499668163815,-12.9649293941461,-12.8797915746879,
-12.7945965012499,-12.7092654850702,-12.6710349417861,-12.5825725222911,
-12.4942230261398,-12.405966583943,-12.3172632542332,-12.2291343186378,
-12.1410336270666,-12.0529433623445,-11.9637925083244,-11.8756388741685,
-11.7859894102163,-11.6963399462641,-11.6077342332092,-11.5191955002859,
-11.4307068279097,-11.342248612659,-11.2537923358304,-11.2089924485031,
-11.1135915257343,-11.0156048819863,-10.9199968256523,-10.8208208881972,
-10.7216449507421,-10.6332463945045,-10.5448975523916,-10.494778244858),
 .UNSPECIFIED.);
#716=B_SPLINE_CURVE_WITH_KNOTS('',3,(#65810,#65811,#65812,#65813,#65814,
#65815,#65816,#65817,#65818,#65819,#65820,#65821,#65822,#65823,#65824,#65825,
#65826,#65827,#65828,#65829,#65830,#65831,#65832,#65833,#65834,#65835,#65836,
#65837,#65838,#65839,#65840,#65841,#65842,#65843,#65844,#65845,#65846,#65847,
#65848,#65849,#65850,#65851,#65852,#65853,#65854,#65855,#65856,#65857,#65858,
#65859,#65860,#65861,#65862,#65863,#65864,#65865,#65866,#65867,#65868,#65869,
#65870,#65871,#65872,#65873,#65874,#65875,#65876,#65877,#65878,#65879,#65880,
#65881,#65882,#65883,#65884,#65885,#65886,#65887,#65888,#65889,#65890,#65891,
#65892,#65893,#65894,#65895,#65896,#65897,#65898,#65899,#65900,#65901,#65902,
#65903,#65904,#65905,#65906,#65907,#65908,#65909,#65910,#65911,#65912,#65913,
#65914,#65915,#65916,#65917,#65918,#65919,#65920,#65921,#65922,#65923,#65924,
#65925,#65926,#65927,#65928,#65929,#65930,#65931,#65932,#65933,#65934,#65935,
#65936,#65937,#65938,#65939,#65940,#65941,#65942,#65943,#65944,#65945,#65946,
#65947,#65948,#65949,#65950,#65951,#65952,#65953,#65954,#65955,#65956,#65957,
#65958,#65959,#65960,#65961,#65962,#65963,#65964,#65965,#65966,#65967,#65968,
#65969,#65970,#65971,#65972,#65973,#65974,#65975,#65976,#65977,#65978,#65979,
#65980,#65981,#65982,#65983,#65984,#65985,#65986,#65987,#65988,#65989,#65990,
#65991,#65992,#65993,#65994,#65995,#65996,#65997,#65998,#65999,#66000,#66001,
#66002,#66003,#66004,#66005,#66006,#66007,#66008,#66009,#66010,#66011,#66012,
#66013,#66014,#66015,#66016,#66017,#66018,#66019,#66020,#66021,#66022,#66023,
#66024,#66025,#66026),.UNSPECIFIED.,.F.,.F.,(4,3,3,3,3,3,3,3,3,3,3,3,3,
3,3,3,3,3,3,3,3,3,3,3,3,3,3,3,3,3,3,3,3,3,3,3,3,3,3,3,3,3,3,3,3,3,3,3,3,
3,3,3,3,3,3,3,3,3,3,3,3,3,3,3,3,3,3,3,3,3,3,3,4),(14.2319032050023,14.3180783398705,
14.4043013520915,14.4905508815598,14.5768909610204,14.6204249328301,14.7090317212767,
14.7975715349282,14.8860612901713,14.9745205887241,15.0629779437081,15.1077724305911,
15.2031708278285,15.3011581029594,15.3967634736636,15.4959417010079,15.5951199283521,
15.6835192874087,15.7718698144088,15.8601984027851,15.9485126799093,16.0368502402501,
16.0824674261131,16.1752378011632,16.2680191188897,16.3608252586661,16.4536335932026,
16.5464539861204,16.5698149238741,16.6602714687669,16.7507017943729,16.8411292346796,
16.9315506889061,17.0219940616611,17.0571624216351,17.1484889520193,17.2398000990734,
17.3311157956058,17.422427582782,17.5137570989986,17.5445099193961,17.6356082056985,
17.7266885987632,17.8177722450881,17.908851891124,17.9999511154388,18.0318574171571,
18.1229465647275,18.2140172401526,18.3050904133561,18.3961591751174,18.4872470013927,
18.5192049149181,18.6103536567512,18.7014849737903,18.792619714476,18.8837504128207,
18.9749001970642,19.0065524126791,19.0976529191154,19.1887352474846,19.2798203891772,
19.3709012703821,19.4620013365704,19.4938999104401,19.5850275018026,19.6761373102866,
19.7672502347794,19.8583589984622,19.9494868590967,19.9812474082011,20.0749895405449,
20.1579098627142),.UNSPECIFIED.);
#717=B_SPLINE_CURVE_WITH_KNOTS('',3,(#66027,#66028,#66029,#66030,#66031,
#66032,#66033,#66034,#66035,#66036,#66037,#66038,#66039,#66040,#66041,#66042),
 .UNSPECIFIED.,.F.,.F.,(4,3,3,3,3,4),(20.1579098629397,20.2491418453206,
20.3403708768365,20.4316208898443,20.4685949059621,20.5146317045532),
 .UNSPECIFIED.);
#718=B_SPLINE_CURVE_WITH_KNOTS('',3,(#66049,#66050,#66051,#66052,#66053,
#66054,#66055,#66056,#66057,#66058,#66059,#66060,#66061,#66062),
 .UNSPECIFIED.,.F.,.F.,(4,2,2,2,2,2,4),(-3.36831712780366,-3.29736812950927,
-3.2281135588852,-3.10483059742013,-3.02255231766649,-2.85213247050082,
-2.84070125419267),.UNSPECIFIED.);
#719=B_SPLINE_CURVE_WITH_KNOTS('',3,(#66069,#66070,#66071,#66072,#66073,
#66074,#66075,#66076,#66077,#66078,#66079,#66080,#66081,#66082),
 .UNSPECIFIED.,.F.,.F.,(4,2,2,2,2,2,4),(-3.36831719559857,-3.29736749922203,
-3.22811229767945,-3.10483036543586,-3.02255213049028,-2.85213226983663,
-2.84070132266613),.UNSPECIFIED.);
#720=B_SPLINE_CURVE_WITH_KNOTS('',3,(#66088,#66089,#66090,#66091,#66092,
#66093,#66094,#66095,#66096,#66097,#66098,#66099,#66100,#66101,#66102,#66103,
#66104,#66105,#66106,#66107,#66108,#66109,#66110,#66111,#66112,#66113,#66114,
#66115,#66116,#66117,#66118,#66119,#66120,#66121,#66122,#66123,#66124,#66125,
#66126,#66127,#66128,#66129,#66130,#66131,#66132,#66133,#66134,#66135,#66136,
#66137,#66138,#66139,#66140,#66141,#66142,#66143,#66144,#66145,#66146,#66147,
#66148,#66149,#66150,#66151,#66152,#66153,#66154,#66155,#66156,#66157,#66158,
#66159,#66160,#66161,#66162,#66163,#66164,#66165,#66166,#66167,#66168,#66169,
#66170,#66171,#66172,#66173,#66174,#66175,#66176,#66177,#66178,#66179,#66180,
#66181,#66182,#66183,#66184,#66185,#66186,#66187,#66188,#66189,#66190,#66191,
#66192,#66193,#66194,#66195,#66196,#66197,#66198,#66199,#66200,#66201,#66202,
#66203,#66204,#66205,#66206,#66207,#66208,#66209,#66210,#66211,#66212,#66213,
#66214,#66215,#66216,#66217,#66218,#66219,#66220,#66221,#66222,#66223,#66224,
#66225,#66226,#66227,#66228,#66229,#66230,#66231,#66232,#66233,#66234,#66235,
#66236,#66237,#66238,#66239,#66240,#66241,#66242,#66243,#66244,#66245,#66246,
#66247,#66248,#66249,#66250,#66251,#66252,#66253,#66254,#66255,#66256,#66257,
#66258,#66259,#66260,#66261,#66262,#66263,#66264,#66265,#66266,#66267,#66268,
#66269,#66270,#66271,#66272,#66273,#66274,#66275,#66276,#66277,#66278,#66279,
#66280,#66281,#66282,#66283,#66284,#66285,#66286,#66287,#66288,#66289,#66290,
#66291,#66292,#66293,#66294,#66295,#66296,#66297,#66298,#66299,#66300,#66301),
 .UNSPECIFIED.,.F.,.F.,(4,3,3,3,3,3,3,3,3,3,3,3,3,3,3,3,3,3,3,3,3,3,3,3,
3,3,3,3,3,3,3,3,3,3,3,3,3,3,3,3,3,3,3,3,3,3,3,3,3,3,3,3,3,3,3,3,3,3,3,3,
3,3,3,3,3,3,3,3,3,3,3,4),(20.5146317059255,20.6057411556705,20.6968512036646,
20.787952699175,20.8790768172452,20.9559424037231,21.0470612884176,21.1381622711603,
21.2292662844587,21.3203661118309,21.4114850745217,21.4432899014841,21.5344090077396,
21.6255102062777,21.7166144247242,21.8077144504978,21.8988336000398,21.9306373992451,
22.0217552919853,22.1128552791001,22.2039583013779,22.2950571431046,22.3861751362555,
22.4179848970061,22.509105908084,22.6002090175663,22.6913151367396,22.7824170521249,
22.8735380592111,22.9053323947671,22.9964483149354,23.0875463288368,23.1786473967051,
23.2697443002416,23.3608603950902,23.3926798925281,23.4838001230218,23.5749024336183,
23.6660077353362,23.7571088247932,23.8482290006467,23.8800273902891,23.9711543961236,
24.0622635601542,24.1533757600712,24.2444837545981,24.3356107871391,24.3673748880501,
24.4584574255276,24.5495218955094,24.6405895201973,24.7316531300112,24.8227364288934,
24.8547223858112,24.9459388473859,25.0371377774975,25.1283392870914,25.2195360775557,
25.3107504070892,25.3420698835721,25.4329781236218,25.5238682415749,25.6147631576547,
25.7056554643935,25.7965709429544,25.8294173813331,25.9210354533695,26.012634445065,
26.1042294234823,26.1958146217395,26.2874065688899,26.3167648790942),
 .UNSPECIFIED.);
#721=B_SPLINE_CURVE_WITH_KNOTS('',3,(#66303,#66304,#66305,#66306,#66307,
#66308,#66309,#66310,#66311,#66312,#66313,#66314,#66315,#66316,#66317,#66318,
#66319,#66320,#66321,#66322,#66323,#66324,#66325,#66326,#66327,#66328,#66329,
#66330,#66331,#66332,#66333,#66334,#66335,#66336,#66337,#66338,#66339,#66340,
#66341,#66342,#66343,#66344,#66345,#66346,#66347,#66348,#66349,#66350,#66351,
#66352,#66353,#66354,#66355,#66356),.UNSPECIFIED.,.F.,.F.,(4,2,2,2,2,2,
2,2,2,2,2,2,2,2,2,2,2,2,2,2,2,2,2,2,2,2,4),(-2.84070132266613,-2.78020515581023,
-2.65435156006841,-2.57658993540392,-2.49698956383074,-2.32946341040136,
-2.24549532116482,-2.17252610320999,-2.05532975785649,-1.97398058008043,
-1.85252492978697,-1.68460878885054,-1.51626217315707,-1.44268575556167,
-1.30223153656894,-1.22322211388899,-1.10079068218151,-1.03028045314551,
-0.859935588437529,-0.777911177383843,-0.65632125055536,-0.575111733431278,
-0.460088756394275,-0.393765504197562,-0.309841478073698,-0.154378575284087,
-0.153225086960603),.UNSPECIFIED.);
#722=B_SPLINE_CURVE_WITH_KNOTS('',3,(#66362,#66363,#66364,#66365,#66366,
#66367,#66368,#66369,#66370,#66371,#66372,#66373,#66374,#66375,#66376,#66377,
#66378,#66379,#66380,#66381,#66382,#66383,#66384,#66385,#66386,#66387,#66388,
#66389,#66390,#66391,#66392,#66393,#66394,#66395,#66396,#66397,#66398,#66399,
#66400,#66401,#66402,#66403,#66404,#66405,#66406,#66407,#66408,#66409,#66410,
#66411,#66412,#66413,#66414,#66415,#66416,#66417,#66418,#66419,#66420,#66421,
#66422,#66423,#66424,#66425,#66426,#66427,#66428,#66429,#66430,#66431,#66432,
#66433,#66434,#66435,#66436,#66437,#66438,#66439,#66440,#66441,#66442,#66443,
#66444,#66445,#66446,#66447,#66448,#66449,#66450,#66451,#66452,#66453,#66454,
#66455,#66456,#66457,#66458,#66459,#66460,#66461,#66462,#66463,#66464,#66465,
#66466,#66467,#66468,#66469,#66470,#66471,#66472,#66473,#66474,#66475,#66476,
#66477,#66478,#66479,#66480,#66481,#66482,#66483,#66484,#66485,#66486,#66487,
#66488,#66489,#66490,#66491,#66492,#66493,#66494,#66495,#66496,#66497,#66498,
#66499,#66500,#66501,#66502,#66503,#66504,#66505,#66506,#66507,#66508,#66509,
#66510,#66511,#66512,#66513,#66514,#66515,#66516,#66517,#66518,#66519,#66520,
#66521,#66522,#66523,#66524,#66525,#66526,#66527,#66528,#66529,#66530,#66531,
#66532,#66533,#66534,#66535,#66536,#66537,#66538,#66539,#66540,#66541,#66542,
#66543,#66544,#66545,#66546,#66547,#66548,#66549,#66550,#66551,#66552,#66553,
#66554,#66555,#66556,#66557,#66558,#66559,#66560,#66561,#66562,#66563,#66564,
#66565,#66566,#66567,#66568,#66569,#66570,#66571,#66572,#66573,#66574,#66575,
#66576,#66577,#66578),.UNSPECIFIED.,.F.,.F.,(4,3,3,3,3,3,3,3,3,3,3,3,3,
3,3,3,3,3,3,3,3,3,3,3,3,3,3,3,3,3,3,3,3,3,3,3,3,3,3,3,3,3,3,3,3,3,3,3,3,
3,3,3,3,3,3,3,3,3,3,3,3,3,3,3,3,3,3,3,3,3,3,3,4),(14.2319029117468,14.3180786703085,
14.4043023140868,14.4905524798541,14.5768932001375,14.6204249328301,14.709029072133,
14.7975662235017,14.8860533112043,14.9745099411476,15.0629646402058,15.1077724305911,
15.2031770525732,15.301162771518,15.3967747615889,15.4959473449705,15.5951199283521,
15.6835147693779,15.7718607477815,15.8601847664223,15.9484944641987,16.0368274563183,
16.0824674261131,16.1752416501605,16.2680268918029,16.3608370085562,16.4536493321215,
16.5464736883574,16.5698149238741,16.6602697202645,16.7506982784102,16.8411239387326,
16.9315436094234,17.02198520695,17.0571624216351,17.1484896189004,17.2398014408522,
17.3311178169076,17.4224302842788,17.513760475784,17.5445099193961,17.6356081111592,
17.7266884093325,17.8177719612098,17.9088515133148,17.9999506452483,18.0318574171571,
18.1229464656923,18.2140170402529,18.3050901109109,18.3961587694273,18.4872464922916,
18.5192049149181,18.6103537750563,18.7014852122315,18.7926200745213,18.8837508949863,
18.9749008010787,19.0065524126791,19.0976528378301,19.1887350837563,19.2798201421328,
19.370900939742,19.4620009226222,19.4938999104401,19.585027544216,19.6761373956887,
19.7672503635792,19.8583591707788,19.9494870747378,19.9812474082011,20.074989510816,
20.1579098627142),.UNSPECIFIED.);
#723=B_SPLINE_CURVE_WITH_KNOTS('',3,(#66579,#66580,#66581,#66582,#66583,
#66584,#66585,#66586,#66587,#66588,#66589,#66590,#66591,#66592,#66593,#66594),
 .UNSPECIFIED.,.F.,.F.,(4,3,3,3,3,4),(20.1579098629397,20.2491418336797,
20.3403708535511,20.4316208550079,20.4685949059621,20.5146317059255),
 .UNSPECIFIED.);
#724=B_SPLINE_CURVE_WITH_KNOTS('',3,(#66596,#66597,#66598,#66599,#66600,
#66601),.UNSPECIFIED.,.F.,.F.,(4,2,4),(-0.153225086960603,-0.0778068263849535,
-0.000838734811037899),.UNSPECIFIED.);
#725=B_SPLINE_CURVE_WITH_KNOTS('',3,(#66602,#66603,#66604,#66605,#66606,
#66607,#66608,#66609,#66610,#66611,#66612,#66613,#66614,#66615,#66616,#66617,
#66618,#66619,#66620,#66621,#66622,#66623,#66624,#66625,#66626,#66627,#66628,
#66629,#66630,#66631,#66632,#66633,#66634,#66635,#66636,#66637,#66638,#66639,
#66640,#66641,#66642,#66643,#66644,#66645,#66646,#66647,#66648,#66649,#66650,
#66651,#66652,#66653,#66654,#66655,#66656,#66657,#66658,#66659,#66660,#66661,
#66662,#66663,#66664,#66665,#66666,#66667,#66668,#66669,#66670,#66671,#66672,
#66673,#66674,#66675,#66676,#66677,#66678,#66679,#66680,#66681,#66682,#66683,
#66684,#66685,#66686,#66687,#66688,#66689,#66690,#66691,#66692,#66693,#66694,
#66695,#66696,#66697,#66698,#66699,#66700,#66701,#66702,#66703,#66704,#66705,
#66706,#66707,#66708,#66709,#66710,#66711,#66712,#66713,#66714,#66715,#66716,
#66717,#66718,#66719,#66720,#66721,#66722,#66723,#66724,#66725,#66726,#66727,
#66728,#66729,#66730,#66731,#66732,#66733,#66734,#66735,#66736,#66737,#66738,
#66739,#66740,#66741,#66742,#66743,#66744,#66745,#66746,#66747,#66748,#66749,
#66750,#66751,#66752,#66753,#66754,#66755,#66756,#66757,#66758,#66759,#66760,
#66761,#66762,#66763,#66764,#66765,#66766,#66767,#66768,#66769,#66770,#66771,
#66772,#66773,#66774,#66775,#66776,#66777,#66778,#66779,#66780,#66781,#66782,
#66783,#66784,#66785,#66786,#66787,#66788,#66789,#66790,#66791,#66792,#66793,
#66794,#66795,#66796,#66797,#66798,#66799,#66800,#66801,#66802,#66803,#66804,
#66805,#66806,#66807,#66808,#66809),.UNSPECIFIED.,.F.,.F.,(4,3,3,3,3,3,
3,3,3,3,3,3,3,3,3,3,3,3,3,3,3,3,3,3,3,3,3,3,3,3,3,3,3,3,3,3,3,3,3,3,3,3,
3,3,3,3,3,3,3,3,3,3,3,3,3,3,3,3,3,3,3,3,3,3,3,3,3,3,3,4),(-16.4213910178811,
-16.3286400772641,-16.2359063591921,-16.1431843748859,-16.0824674261131,
-15.9941362568266,-15.9058273801709,-15.8175005869686,-15.7291653788733,
-15.6407726083022,-15.5951199283521,-15.4994633914501,-15.4015406512354,
-15.3059593709262,-15.2068659007586,-15.1077724305911,-15.0193205338912,
-14.9308712775328,-14.84237561715,-14.7538553588308,-14.6652542472042,-14.6204249328301,
-14.5321659202474,-14.4439801271102,-14.3558478376921,-14.2670831001441,
-14.1789808129682,-14.0908700658319,-14.0027330472036,-13.9134822697297,
-13.8251919559008,-13.7354609466044,-13.6457299373081,-13.5603976716426,
-13.4751811547976,-13.390056640956,-13.3050005048409,-13.2199799188415,
-13.1349748337167,-13.0499640026098,-12.9649261753039,-12.8797879523774,
-12.7945924756304,-12.7092610599517,-12.6710349417861,-12.5825724970548,
-12.4942229702032,-12.4059664919653,-12.3172631737526,-12.2291341894402,
-12.1410334445326,-12.0529431219476,-11.9637923280267,-11.8756386254687,
-11.7859892858664,-11.6963399462641,-11.6077363315675,-11.5191997074042,
-11.430713147944,-11.3422570464542,-11.253802873335,-11.2089924485031,-11.1135865925285,
-11.0156011820819,-10.9199878797788,-10.8208164152605,-10.7216449507421,
-10.6332499745261,-10.5449047398611,-10.49477808198),.UNSPECIFIED.);
#726=B_SPLINE_CURVE_WITH_KNOTS('',3,(#66815,#66816,#66817,#66818,#66819,
#66820,#66821,#66822,#66823,#66824,#66825,#66826,#66827,#66828,#66829,#66830,
#66831,#66832,#66833,#66834,#66835,#66836,#66837,#66838,#66839,#66840,#66841,
#66842,#66843,#66844,#66845,#66846,#66847,#66848,#66849,#66850,#66851,#66852),
 .UNSPECIFIED.,.F.,.F.,(4,2,2,2,2,2,2,2,2,2,2,2,2,2,2,2,2,2,4),(2.08228018305572E-5,
0.134148024868073,0.202716477712664,0.327559837231032,0.405484389532305,
0.485128229324024,0.652510410323932,0.736487383617962,0.809797659300728,
0.977479155573237,1.04684058460045,1.11942531708603,1.23168220985833,1.31165597792338,
1.44944632348465,1.58444765771081,1.65977704604661,1.79047000383681,1.80129261558726),
 .UNSPECIFIED.);
#727=B_SPLINE_CURVE_WITH_KNOTS('',3,(#66856,#66857,#66858,#66859,#66860,
#66861,#66862,#66863,#66864,#66865,#66866,#66867,#66868,#66869,#66870),
 .UNSPECIFIED.,.F.,.F.,(4,1,1,1,1,1,1,1,1,1,1,1,4),(2.0217817672715,2.43673748880501,
2.92408498656602,3.41143248432702,3.89877998208802,4.38612747984903,4.87347497761003,
5.36082247537103,5.84816997313203,6.33551747089303,6.82286496865404,7.31021246641504,
7.59153924858053),.UNSPECIFIED.);
#728=B_SPLINE_CURVE_WITH_KNOTS('',3,(#66871,#66872,#66873,#66874,#66875,
#66876,#66877,#66878,#66879,#66880,#66881,#66882,#66883,#66884,#66885,#66886),
 .UNSPECIFIED.,.F.,.F.,(4,3,3,3,3,4),(7.59153924858053,7.68452254538593,
7.77753312315858,7.79755996417604,7.88865003464089,7.94826257357117),
 .UNSPECIFIED.);
#729=B_SPLINE_CURVE_WITH_KNOTS('',3,(#66892,#66893,#66894,#66895,#66896,
#66897,#66898,#66899,#66900,#66901,#66902,#66903,#66904,#66905,#66906,#66907,
#66908,#66909,#66910,#66911,#66912,#66913,#66914,#66915,#66916,#66917),
 .UNSPECIFIED.,.F.,.F.,(4,2,2,2,2,2,2,2,2,2,2,2,4),(-0.0747573509028117,
-0.0739383148717887,-0.0616383873536828,-0.0559544033060534,-0.0377854288912249,
-0.0350633930401213,-0.0337175069903932,-0.0326484285706749,-0.0316335607138953,
-0.0303960629492908,-0.0285520710439741,-0.0215326227016456,-0.000655565290617223),
 .UNSPECIFIED.);
#730=B_SPLINE_CURVE_WITH_KNOTS('',3,(#66919,#66920,#66921,#66922,#66923,
#66924,#66925,#66926,#66927,#66928,#66929,#66930,#66931,#66932,#66933,#66934,
#66935,#66936,#66937,#66938,#66939,#66940,#66941,#66942,#66943,#66944,#66945,
#66946,#66947,#66948,#66949,#66950,#66951,#66952,#66953,#66954,#66955,#66956,
#66957,#66958,#66959,#66960,#66961,#66962,#66963,#66964,#66965,#66966,#66967,
#66968,#66969,#66970,#66971,#66972,#66973,#66974,#66975,#66976,#66977,#66978,
#66979,#66980,#66981,#66982,#66983,#66984,#66985,#66986,#66987,#66988,#66989,
#66990,#66991,#66992,#66993,#66994,#66995,#66996,#66997,#66998,#66999,#67000,
#67001,#67002,#67003,#67004,#67005,#67006,#67007,#67008,#67009,#67010,#67011,
#67012,#67013,#67014,#67015,#67016,#67017,#67018,#67019,#67020,#67021,#67022,
#67023,#67024,#67025,#67026,#67027,#67028,#67029,#67030,#67031,#67032,#67033,
#67034,#67035,#67036),.UNSPECIFIED.,.F.,.F.,(4,3,3,3,3,3,3,3,3,3,3,3,3,
3,3,3,3,3,3,3,3,3,3,3,3,3,3,3,3,3,3,3,3,3,3,3,3,3,3,4),(170.955339710339,
171.060905920727,171.162663401337,171.264353092419,171.366010725341,171.467671982924,
171.569433774829,171.671256091623,171.77323959999,171.799869393442,171.903390623982,
172.006760853885,172.110012748576,172.2132010018,172.316359435341,172.419521829469,
172.522792194405,172.626119678124,172.729629765827,172.798705843404,172.90100919765,
173.00315849853,173.10519039517,173.207159585109,173.309101433958,173.411051266852,
173.513123449993,173.615258630591,173.71759950971,173.797542293366,173.903815983742,
174.01538632869,174.121306695383,174.227127466107,174.332876381024,174.438581090584,
174.544298932523,174.650021856933,174.755817740451,174.796378743328),
 .UNSPECIFIED.);
#731=B_SPLINE_CURVE_WITH_KNOTS('',3,(#67040,#67041,#67042,#67043,#67044,
#67045,#67046,#67047,#67048,#67049,#67050,#67051,#67052,#67053,#67054,#67055,
#67056,#67057,#67058,#67059,#67060,#67061,#67062,#67063,#67064,#67065,#67066,
#67067,#67068,#67069,#67070,#67071,#67072,#67073,#67074,#67075,#67076,#67077,
#67078,#67079,#67080,#67081,#67082,#67083,#67084,#67085,#67086,#67087,#67088,
#67089,#67090,#67091,#67092,#67093,#67094,#67095,#67096,#67097,#67098,#67099,
#67100,#67101,#67102,#67103,#67104,#67105,#67106,#67107,#67108,#67109,#67110,
#67111,#67112,#67113,#67114,#67115,#67116,#67117,#67118,#67119,#67120,#67121,
#67122,#67123,#67124,#67125,#67126,#67127,#67128,#67129,#67130,#67131,#67132,
#67133,#67134,#67135,#67136,#67137,#67138,#67139,#67140,#67141,#67142,#67143,
#67144,#67145,#67146,#67147,#67148,#67149,#67150,#67151,#67152,#67153,#67154,
#67155,#67156,#67157,#67158,#67159,#67160,#67161,#67162,#67163,#67164,#67165,
#67166,#67167,#67168,#67169,#67170,#67171,#67172,#67173,#67174,#67175,#67176,
#67177,#67178,#67179,#67180,#67181,#67182,#67183,#67184,#67185,#67186,#67187,
#67188,#67189,#67190,#67191,#67192,#67193,#67194,#67195,#67196,#67197,#67198,
#67199,#67200,#67201,#67202,#67203,#67204,#67205,#67206,#67207,#67208),
 .UNSPECIFIED.,.F.,.F.,(4,3,3,3,3,3,3,3,3,3,3,3,3,3,3,3,3,3,3,3,3,3,3,3,
3,3,3,3,3,3,3,3,3,3,3,3,3,3,3,3,3,3,3,3,3,3,3,3,3,3,3,3,3,3,3,3,4),(-172.787594226351,
-172.684274645609,-172.581108473843,-172.478063715916,-172.375084159336,
-172.272135658752,-172.169184111836,-172.066127763492,-171.963014418944,
-171.859724811317,-171.799869393442,-171.696296400939,-171.592873101958,
-171.489566394852,-171.386322278747,-171.283106998388,-171.179886839023,
-171.076557646842,-170.973170650988,-170.869600563122,-170.801032943481,
-170.69777070211,-170.594663824546,-170.491680473781,-170.388763813606,
-170.285879610087,-170.182993673711,-170.080001243854,-169.976952951891,
-169.873720941887,-169.802196493519,-169.698775124036,-169.595507109046,
-169.492360393262,-169.389279078215,-169.286229166357,-169.183176703332,
-169.080017631391,-168.976802370632,-168.873404720303,-168.803360043557,
-168.699944496997,-168.596681938659,-168.493540101833,-168.39046330706,
-168.287417549124,-168.184368865631,-168.081212965654,-167.978000541589,
-167.874605151471,-167.804523593595,-167.699671773339,-167.594987964963,
-167.490464903685,-167.386036670661,-167.281667151101,-167.203857020092),
 .UNSPECIFIED.);
#732=B_SPLINE_CURVE_WITH_KNOTS('',3,(#67209,#67210,#67211,#67212,#67213,
#67214,#67215,#67216),.UNSPECIFIED.,.F.,.F.,(4,2,2,4),(-2.66727759453781,
-2.64513467794962,-2.59594303077105,-2.59308707914317),.UNSPECIFIED.);
#733=B_SPLINE_CURVE_WITH_KNOTS('',3,(#67221,#67222,#67223,#67224,#67225,
#67226,#67227,#67228,#67229,#67230,#67231,#67232,#67233,#67234,#67235,#67236,
#67237,#67238,#67239,#67240,#67241,#67242,#67243,#67244,#67245,#67246,#67247,
#67248,#67249,#67250,#67251,#67252,#67253,#67254,#67255,#67256,#67257,#67258,
#67259,#67260,#67261,#67262,#67263,#67264,#67265,#67266,#67267,#67268,#67269,
#67270,#67271,#67272,#67273,#67274,#67275,#67276,#67277,#67278,#67279,#67280,
#67281,#67282,#67283,#67284,#67285,#67286,#67287,#67288,#67289,#67290,#67291,
#67292,#67293,#67294,#67295,#67296,#67297,#67298,#67299,#67300,#67301,#67302,
#67303,#67304,#67305,#67306,#67307,#67308,#67309,#67310,#67311,#67312,#67313,
#67314,#67315,#67316,#67317,#67318,#67319,#67320,#67321,#67322,#67323,#67324,
#67325,#67326,#67327,#67328,#67329,#67330,#67331,#67332,#67333,#67334,#67335,
#67336,#67337,#67338,#67339,#67340,#67341,#67342,#67343,#67344,#67345,#67346,
#67347,#67348,#67349,#67350,#67351,#67352,#67353,#67354,#67355,#67356,#67357,
#67358,#67359,#67360,#67361,#67362,#67363,#67364,#67365,#67366,#67367,#67368,
#67369,#67370,#67371,#67372,#67373,#67374,#67375,#67376,#67377,#67378,#67379,
#67380,#67381,#67382,#67383,#67384,#67385,#67386,#67387,#67388,#67389,#67390,
#67391,#67392,#67393,#67394,#67395,#67396,#67397,#67398,#67399,#67400,#67401,
#67402,#67403,#67404,#67405,#67406,#67407,#67408,#67409,#67410,#67411,#67412,
#67413,#67414,#67415,#67416,#67417,#67418,#67419,#67420,#67421,#67422,#67423,
#67424,#67425,#67426,#67427,#67428,#67429,#67430,#67431,#67432,#67433,#67434,
#67435,#67436,#67437,#67438,#67439,#67440,#67441,#67442,#67443,#67444,#67445,
#67446),.UNSPECIFIED.,.F.,.F.,(4,2,2,2,2,2,2,2,2,2,2,2,2,2,2,2,2,2,2,2,
2,2,2,2,2,2,2,2,2,2,2,2,2,2,2,2,2,2,2,2,2,2,2,2,2,2,2,2,2,2,2,2,2,2,2,2,
2,2,2,2,2,2,2,2,2,2,2,2,2,2,2,2,2,2,2,2,2,2,2,2,2,2,2,2,2,2,2,2,2,2,2,2,
2,2,2,2,2,2,2,2,2,2,2,2,2,2,2,2,2,2,2,2,4),(-1.40817977626643,-1.40705404837906,
-1.40292854648138,-1.3757426548093,-1.3337320464292,-1.32763512392359,-1.30978754890451,
-1.30709916425526,-1.30573723566938,-1.30466495450943,-1.30341928540201,
-1.30119586266891,-1.29070305773952,-1.26784056942761,-1.21011170611799,
-1.20367843769144,-1.20117007693688,-1.19935221924447,-1.19740892849055,
-1.19480672238284,-1.1889830009617,-1.16514966199108,-1.11614970333744,
-1.09779132445287,-1.09505198420995,-1.09369779480841,-1.09262569366162,
-1.09137327576406,-1.08912117532948,-1.07817666003123,-1.05366046115555,
-0.998557418932194,-0.991850218090042,-0.98929760171817,-0.987467733874629,
-0.98553005735288,-0.982966800167927,-0.977359065828194,-0.92907584220918,
-0.888723738506282,-0.884011345098199,-0.882271365568769,-0.881246080095021,
-0.880154646224944,-0.878645357309653,-0.875062863423288,-0.870037787607825,
-0.856214116460312,-0.83386094240738,-0.787184939428978,-0.779989395426667,
-0.777074388953639,-0.775273873406327,-0.773322052655055,-0.770660422919828,
-0.764492409594996,-0.737950196320098,-0.698622945036696,-0.687289264474059,
-0.673503769726914,-0.671211303564944,-0.669826550081623,-0.668750098233928,
-0.667534982181281,-0.665449708224016,-0.656908941372315,-0.64035066459171,
-0.598278958259621,-0.571099348034574,-0.566971801379125,-0.564478971054942,
-0.562545228654309,-0.560449567398847,-0.557102065583082,-0.54590445943643,
-0.527329550124218,-0.484797482353254,-0.462028184514635,-0.459170491849498,
-0.457791868994825,-0.456715605017749,-0.455474595675706,-0.453286877187307,
-0.443433219831685,-0.394231943383457,-0.359839415981377,-0.355551723858008,
-0.353009728095418,-0.351065351000036,-0.348985053513911,-0.345718999305572,
-0.335297147001225,-0.318505182775914,-0.258883353406481,-0.249294266218978,
-0.247244927429815,-0.24591830870456,-0.244851270525529,-0.243841554781177,
-0.241869173859128,-0.234451256057864,-0.220918078416166,-0.19233797325591,
-0.147271569436308,-0.143024766803768,-0.140506708098782,-0.138580709949515,
-0.136520279126182,-0.133286131263482,-0.122977226377692,-0.106384758650064,
-0.0845186243735332,-0.0747573509028117),.UNSPECIFIED.);
#734=B_SPLINE_CURVE_WITH_KNOTS('',3,(#67447,#67448,#67449,#67450,#67451,
#67452,#67453,#67454,#67455,#67456,#67457,#67458,#67459,#67460,#67461,#67462,
#67463,#67464,#67465,#67466,#67467,#67468,#67469,#67470,#67471,#67472,#67473,
#67474,#67475,#67476,#67477,#67478,#67479,#67480,#67481,#67482,#67483,#67484,
#67485,#67486,#67487,#67488,#67489,#67490,#67491,#67492,#67493,#67494,#67495,
#67496,#67497,#67498,#67499,#67500,#67501,#67502,#67503,#67504,#67505,#67506,
#67507,#67508,#67509,#67510,#67511,#67512,#67513,#67514,#67515,#67516,#67517,
#67518,#67519,#67520,#67521,#67522,#67523,#67524,#67525,#67526,#67527,#67528,
#67529,#67530,#67531,#67532,#67533,#67534,#67535,#67536,#67537,#67538,#67539,
#67540,#67541,#67542,#67543,#67544,#67545,#67546,#67547,#67548,#67549,#67550,
#67551,#67552,#67553,#67554,#67555,#67556,#67557,#67558,#67559,#67560,#67561,
#67562,#67563,#67564,#67565,#67566,#67567,#67568,#67569,#67570,#67571,#67572,
#67573,#67574,#67575,#67576,#67577,#67578,#67579,#67580,#67581,#67582,#67583,
#67584,#67585,#67586,#67587,#67588,#67589,#67590,#67591,#67592,#67593,#67594,
#67595,#67596,#67597,#67598,#67599,#67600,#67601,#67602,#67603,#67604,#67605,
#67606,#67607,#67608,#67609,#67610,#67611,#67612,#67613,#67614,#67615,#67616,
#67617,#67618,#67619,#67620,#67621,#67622,#67623,#67624,#67625,#67626,#67627,
#67628,#67629,#67630,#67631,#67632,#67633,#67634,#67635,#67636,#67637,#67638,
#67639,#67640,#67641,#67642,#67643,#67644,#67645,#67646,#67647,#67648,#67649,
#67650,#67651,#67652,#67653,#67654,#67655,#67656,#67657,#67658,#67659,#67660,
#67661,#67662,#67663,#67664,#67665,#67666,#67667,#67668,#67669,#67670,#67671,
#67672,#67673,#67674,#67675,#67676,#67677,#67678,#67679,#67680,#67681,#67682,
#67683,#67684,#67685,#67686),.UNSPECIFIED.,.F.,.F.,(4,2,2,2,2,2,2,2,2,2,
2,2,2,2,2,2,2,2,2,2,2,2,2,2,2,2,2,2,2,2,2,2,2,2,2,2,2,2,2,2,2,2,2,2,2,2,
2,2,2,2,2,2,2,2,2,2,2,2,2,2,2,2,2,2,2,2,2,2,2,2,2,2,2,2,2,2,2,2,2,2,2,2,
2,2,2,2,2,2,2,2,2,2,2,2,2,2,2,2,2,2,2,2,2,2,2,2,2,2,2,2,2,2,2,2,2,2,2,2,
2,4),(-2.59308707914317,-2.58660339095032,-2.58445919195256,-2.58323177533603,
-2.58215751868089,-2.58077043530716,-2.57786397952892,-2.55018880910383,
-2.51342558454827,-2.49426240188725,-2.48668611853075,-2.48276630063086,
-2.47946214186469,-2.47740892179214,-2.47557482273063,-2.47314289880733,
-2.46930670208162,-2.44885991797817,-2.39982767402896,-2.38317168920143,
-2.37459660300356,-2.37250763718333,-2.37129113892439,-2.37021375841239,
-2.36882821887161,-2.36653549590919,-2.352776798318,-2.34956221923803,-2.30364431015071,
-2.27574252048464,-2.2694060026503,-2.26671390106241,-2.26475530302475,
-2.26295934469996,-2.26007554580225,-2.25307603892048,-2.20166204145705,
-2.17457501360255,-2.16297249090162,-2.1606835625134,-2.15942370522108,
-2.15835287954249,-2.15701016563937,-2.15441100969585,-2.13887685921022,
-2.13224538774638,-2.11843770774554,-2.08555660440661,-2.06900013269377,
-2.05869293340974,-2.05544501071139,-2.05337209491736,-2.0514317309228,
-2.04889087994364,-2.04459622664776,-2.00945889627829,-1.96051823719871,
-1.95080595205933,-1.94863405103307,-1.9473997476301,-1.94632596381445,
-1.94494745533952,-1.94208504331836,-1.9187250304066,-1.90642929072587,
-1.8735610181683,-1.85702171008859,-1.84672167402945,-1.84347406604569,
-1.8414008763816,-1.83945991991007,-1.83691780450014,-1.83261990550126,
-1.79727828371102,-1.7481056860041,-1.73878848869331,-1.73664401139367,
-1.73541553172288,-1.73434063280646,-1.73295243648934,-1.73004063366615,
-1.69799462154211,-1.66509896851337,-1.64627173589911,-1.63878733585992,
-1.6331650344244,-1.63059944363341,-1.62866178266993,-1.62683325088112,
-1.62428463486109,-1.61760105385288,-1.56220871125131,-1.53786714397332,
-1.52696845967853,-1.52471985742216,-1.52346857113848,-1.52239665890621,
-1.52104187455343,-1.51838773260031,-1.5015054258139,-1.48271832796275,
-1.44975300002144,-1.43310009018563,-1.42274853775617,-1.41949490171918,
-1.41742031456669,-1.41547977023576,-1.41294067605154,-1.40865344674532,
-1.36489353865936,-1.3338431236361,-1.31579288364011,-1.31309721063966,
-1.31173353935863,-1.31066089516692,-1.30941595854817,-1.30719660708235,
-1.29677323663359,-1.27415949578997,-1.25967545240964),.UNSPECIFIED.);
#735=B_SPLINE_CURVE_WITH_KNOTS('',3,(#67692,#67693,#67694,#67695),
 .UNSPECIFIED.,.F.,.F.,(4,4),(158.039785833466,158.388969095546),
 .UNSPECIFIED.);
#736=B_SPLINE_CURVE_WITH_KNOTS('',3,(#67696,#67697,#67698,#67699,#67700,
#67701,#67702,#67703,#67704,#67705,#67706,#67707,#67708,#67709,#67710,#67711,
#67712,#67713,#67714,#67715,#67716,#67717,#67718,#67719,#67720,#67721,#67722,
#67723,#67724,#67725,#67726,#67727,#67728,#67729,#67730,#67731,#67732,#67733,
#67734,#67735,#67736,#67737,#67738,#67739,#67740,#67741,#67742,#67743,#67744,
#67745,#67746,#67747,#67748,#67749,#67750,#67751,#67752,#67753,#67754,#67755,
#67756,#67757,#67758,#67759,#67760,#67761,#67762,#67763,#67764,#67765,#67766,
#67767,#67768,#67769,#67770,#67771,#67772,#67773,#67774,#67775,#67776,#67777,
#67778,#67779,#67780,#67781,#67782,#67783,#67784,#67785,#67786,#67787,#67788,
#67789,#67790,#67791,#67792,#67793,#67794,#67795,#67796,#67797,#67798,#67799,
#67800,#67801,#67802,#67803,#67804,#67805,#67806,#67807,#67808,#67809,#67810,
#67811,#67812,#67813,#67814,#67815,#67816,#67817,#67818,#67819,#67820,#67821,
#67822,#67823,#67824,#67825,#67826,#67827,#67828,#67829,#67830,#67831,#67832,
#67833,#67834,#67835,#67836,#67837,#67838,#67839,#67840,#67841,#67842,#67843,
#67844,#67845,#67846,#67847,#67848,#67849,#67850,#67851,#67852,#67853,#67854,
#67855,#67856,#67857,#67858,#67859,#67860,#67861,#67862,#67863,#67864,#67865,
#67866,#67867,#67868,#67869,#67870,#67871,#67872,#67873,#67874,#67875,#67876,
#67877,#67878,#67879,#67880,#67881,#67882,#67883,#67884,#67885,#67886,#67887,
#67888,#67889,#67890,#67891,#67892,#67893,#67894,#67895,#67896,#67897,#67898,
#67899,#67900,#67901,#67902,#67903,#67904,#67905),.UNSPECIFIED.,.F.,.F.,
(4,2,2,2,2,2,2,2,2,2,2,2,2,2,2,2,2,2,2,2,2,2,2,2,2,2,2,2,2,2,2,2,2,2,2,
2,2,2,2,2,2,2,2,2,2,2,2,2,2,2,2,2,2,2,2,2,2,2,2,2,2,2,2,2,2,2,2,2,2,2,2,
2,2,2,2,2,2,2,2,2,2,2,2,2,2,2,2,2,2,2,2,2,2,2,2,2,2,2,2,2,2,2,2,2,4),(-2.66742168608762,
-2.60891631867856,-2.59007764397007,-2.58078446874693,-2.57864197349874,
-2.57741406063882,-2.57633923786897,-2.57495062526262,-2.57203625467893,
-2.54226133830511,-2.49162589315616,-2.48229452219811,-2.47774260774225,
-2.4750043939937,-2.47252013229421,-2.47064406291432,-2.46881762812438,
-2.46627635089932,-2.4596385901056,-2.40382442043769,-2.37976923285203,
-2.36894807799156,-2.36670434245785,-2.36545420467988,-2.36438230657845,
-2.36302629722187,-2.36088073731076,-2.34984288349558,-2.29863084526714,
-2.26992308987829,-2.2634896846549,-2.2607811211191,-2.25881952762152,-2.25702700783975,
-2.25416222296684,-2.24727819180679,-2.19420894295487,-2.16830014997293,
-2.15699277058606,-2.15472035925147,-2.15346399585151,-2.15239272370896,
-2.1510451002617,-2.14842374276434,-2.13238357857934,-2.12707470228156,
-2.11250761379384,-2.07961726854607,-2.06305114959986,-2.05273923724512,
-2.04949046214227,-2.04741714979941,-2.04547651675621,-2.04293545891172,
-2.03864077531949,-2.00353502978294,-1.95465173086845,-1.94486010336139,
-1.94268253678395,-1.94144686883343,-1.9403731914348,-1.93899644170192,
-1.93614300531494,-1.91344691262992,-1.87272244847054,-1.84568047407998,
-1.83944847022109,-1.83677412701535,-1.83481853110581,-1.83301840721638,
-1.83011261847492,-1.82298231667828,-1.77422753641161,-1.73505269101668,
-1.73147803677481,-1.7299690266759,-1.72887686259395,-1.72785087591977,
-1.72610765891376,-1.72137455777659,-1.68179787421688,-1.63388991451972,
-1.62749311103965,-1.62479053543221,-1.62282984380313,-1.62103578005503,
-1.61816336359812,-1.6112342296848,-1.55875523121196,-1.53242869245377,
-1.52101503560159,-1.51873640346793,-1.51747862048654,-1.5164074474784,
-1.51506158505104,-1.51244823859092,-1.49656822458989,-1.49069798720759,
-1.44666701832739,-1.42810815459567,-1.41691845469197,-1.41357286139829,
-1.41147833564995,-1.40954560842506,-1.40817977626643),.UNSPECIFIED.);
#737=B_SPLINE_CURVE_WITH_KNOTS('',3,(#67907,#67908,#67909,#67910,#67911,
#67912,#67913,#67914,#67915,#67916,#67917,#67918,#67919,#67920,#67921,#67922,
#67923,#67924,#67925,#67926,#67927,#67928,#67929,#67930,#67931,#67932,#67933,
#67934,#67935,#67936,#67937,#67938,#67939,#67940,#67941,#67942,#67943,#67944,
#67945,#67946,#67947,#67948,#67949,#67950,#67951,#67952,#67953,#67954,#67955,
#67956,#67957,#67958,#67959,#67960,#67961,#67962,#67963,#67964,#67965,#67966,
#67967,#67968,#67969,#67970,#67971,#67972,#67973,#67974,#67975,#67976,#67977,
#67978,#67979,#67980,#67981,#67982,#67983,#67984,#67985,#67986,#67987,#67988,
#67989,#67990,#67991,#67992,#67993,#67994,#67995,#67996,#67997,#67998,#67999,
#68000,#68001,#68002,#68003,#68004,#68005,#68006,#68007,#68008,#68009,#68010,
#68011,#68012,#68013,#68014,#68015,#68016,#68017,#68018,#68019,#68020,#68021,
#68022,#68023,#68024,#68025,#68026,#68027,#68028,#68029,#68030,#68031,#68032,
#68033,#68034,#68035,#68036,#68037,#68038,#68039,#68040,#68041,#68042,#68043,
#68044,#68045,#68046,#68047,#68048,#68049,#68050,#68051,#68052,#68053,#68054,
#68055,#68056,#68057,#68058,#68059,#68060,#68061,#68062,#68063,#68064,#68065,
#68066,#68067,#68068,#68069,#68070,#68071,#68072,#68073,#68074,#68075,#68076,
#68077,#68078,#68079,#68080,#68081,#68082,#68083,#68084,#68085,#68086,#68087,
#68088,#68089,#68090,#68091,#68092,#68093,#68094,#68095,#68096,#68097,#68098,
#68099,#68100,#68101,#68102,#68103,#68104,#68105,#68106,#68107,#68108,#68109,
#68110,#68111,#68112,#68113,#68114,#68115,#68116,#68117,#68118,#68119,#68120,
#68121,#68122,#68123,#68124),.UNSPECIFIED.,.F.,.F.,(4,2,2,2,2,2,2,2,2,2,
2,2,2,2,2,2,2,2,2,2,2,2,2,2,2,2,2,2,2,2,2,2,2,2,2,2,2,2,2,2,2,2,2,2,2,2,
2,2,2,2,2,2,2,2,2,2,2,2,2,2,2,2,2,2,2,2,2,2,2,2,2,2,2,2,2,2,2,2,2,2,2,2,
2,2,2,2,2,2,2,2,2,2,2,2,2,2,2,2,2,2,2,2,2,2,2,2,2,2,4),(-1.25967545240964,
-1.21603450062663,-1.20965074388613,-1.20715044527458,-1.20533455736151,
-1.20338974317654,-1.20077919166635,-1.19491004781942,-1.17073316723345,
-1.12024909211881,-1.11981771635252,-1.10363128851434,-1.10100429816945,
-1.09965533242265,-1.09858382112367,-1.09732814791181,-1.0950593759243,
-1.08381930989898,-1.05817324909408,-1.00467041016011,-0.997816279860048,
-0.994956195199608,-0.993164369803906,-0.991201732196623,-0.988488404215831,
-0.982027865896532,-0.928091077431277,-0.891881747497268,-0.889027100044917,
-0.88765004663581,-0.886576260003394,-0.88534061670953,-0.883163442615538,
-0.873379711594447,-0.824459281097766,-0.789336857387192,-0.785041540824683,
-0.782500245766603,-0.780559499431617,-0.778486130777015,-0.775237400962393,
-0.764926665557967,-0.74836570266938,-0.715506838201965,-0.701764290024532,
-0.694918605780388,-0.694617606395491,-0.689272618525284,-0.679046785444263,
-0.676953690046489,-0.675613735928834,-0.674542897810459,-0.6732804504582,
-0.670980060592823,-0.659174101423956,-0.609440981833727,-0.577290998430011,
-0.573047500398641,-0.570521388151345,-0.5685832562753,-0.566503913936642,
-0.563227376669613,-0.552670037094953,-0.535559300082063,-0.490855041937219,
-0.467947985146961,-0.465089509731197,-0.463711842265131,-0.462638156455778,
-0.461403283918996,-0.459229028439546,-0.449484199246655,-0.400540681780043,
-0.365414331604263,-0.361119622900382,-0.358578726476474,-0.356638306991323,
-0.354565309237553,-0.351317205877297,-0.341008839774697,-0.324452044065934,
-0.269353861263425,-0.255460787948246,-0.25316186225543,-0.251774615966507,
-0.250697334644219,-0.249482811132885,-0.247442410732315,-0.239363469070486,
-0.224068135375557,-0.194118069974039,-0.189562252439922,-0.153470226585707,
-0.148747145118772,-0.146324136468359,-0.14440527489037,-0.142252619221595,
-0.138644787576576,-0.124692185510215,-0.0975100746812418,-0.074965690734507,
-0.0441240230176781,-0.0412117859648847,-0.039823666732855,-0.0387489813187693,
-0.0375209610406752,-0.0362288375614461,-0.0342508993908115,-0.000628702460286411),
 .UNSPECIFIED.);
#738=B_SPLINE_CURVE_WITH_KNOTS('',3,(#68125,#68126,#68127,#68128,#68129,
#68130,#68131,#68132,#68133,#68134,#68135,#68136,#68137,#68138,#68139,#68140,
#68141,#68142),.UNSPECIFIED.,.F.,.F.,(4,2,2,2,2,2,2,2,4),(-2.66795380407825,
-2.63770974612478,-2.61100504121503,-2.60481461466704,-2.60214740071707,
-2.60019300038953,-2.59839116228356,-2.59547634001882,-2.59347629365865),
 .UNSPECIFIED.);
#739=B_SPLINE_CURVE_WITH_KNOTS('',3,(#68148,#68149,#68150,#68151,#68152,
#68153,#68154,#68155,#68156,#68157,#68158,#68159,#68160),.UNSPECIFIED.,
 .F.,.F.,(4,3,3,3,4),(151.755345441108,151.823140394205,151.951948597244,
152.078650414019,152.105783788367),.UNSPECIFIED.);
#740=B_SPLINE_CURVE_WITH_KNOTS('',3,(#68161,#68162,#68163,#68164,#68165,
#68166,#68167,#68168,#68169,#68170),.UNSPECIFIED.,.F.,.F.,(4,1,1,1,1,1,
1,4),(152.105783788367,152.821976844167,153.820813294129,154.819649744091,
155.818486194052,156.817322644014,157.816159093976,158.039785833466),
 .UNSPECIFIED.);
#741=B_SPLINE_CURVE_WITH_KNOTS('',3,(#68171,#68172,#68173,#68174,#68175,
#68176,#68177,#68178,#68179,#68180,#68181,#68182,#68183,#68184,#68185,#68186,
#68187,#68188,#68189,#68190,#68191,#68192,#68193,#68194,#68195,#68196,#68197,
#68198,#68199,#68200,#68201,#68202,#68203,#68204,#68205,#68206,#68207,#68208,
#68209,#68210,#68211,#68212,#68213,#68214,#68215,#68216,#68217,#68218,#68219,
#68220,#68221,#68222,#68223,#68224,#68225,#68226,#68227,#68228,#68229,#68230,
#68231,#68232,#68233,#68234,#68235,#68236,#68237,#68238,#68239,#68240,#68241,
#68242,#68243,#68244,#68245,#68246,#68247,#68248,#68249,#68250,#68251,#68252,
#68253,#68254,#68255,#68256,#68257,#68258,#68259,#68260,#68261,#68262,#68263,
#68264,#68265,#68266,#68267,#68268,#68269,#68270,#68271,#68272,#68273,#68274,
#68275,#68276,#68277,#68278,#68279,#68280,#68281,#68282,#68283,#68284,#68285,
#68286,#68287,#68288,#68289,#68290,#68291,#68292,#68293,#68294,#68295,#68296,
#68297,#68298,#68299,#68300,#68301,#68302,#68303,#68304,#68305,#68306,#68307,
#68308,#68309,#68310,#68311,#68312,#68313,#68314,#68315,#68316,#68317,#68318,
#68319,#68320,#68321,#68322,#68323,#68324,#68325,#68326,#68327,#68328,#68329,
#68330,#68331,#68332,#68333,#68334,#68335,#68336,#68337,#68338,#68339,#68340,
#68341,#68342,#68343,#68344,#68345,#68346,#68347,#68348,#68349,#68350,#68351,
#68352,#68353,#68354,#68355,#68356,#68357,#68358,#68359,#68360,#68361,#68362,
#68363,#68364,#68365,#68366,#68367,#68368,#68369,#68370,#68371,#68372,#68373,
#68374,#68375,#68376,#68377,#68378,#68379,#68380,#68381,#68382,#68383,#68384,
#68385,#68386,#68387,#68388,#68389,#68390,#68391,#68392,#68393,#68394,#68395,
#68396,#68397,#68398,#68399,#68400),.UNSPECIFIED.,.F.,.F.,(4,2,2,2,2,2,
2,2,2,2,2,2,2,2,2,2,2,2,2,2,2,2,2,2,2,2,2,2,2,2,2,2,2,2,2,2,2,2,2,2,2,2,
2,2,2,2,2,2,2,2,2,2,2,2,2,2,2,2,2,2,2,2,2,2,2,2,2,2,2,2,2,2,2,2,2,2,2,2,
2,2,2,2,2,2,2,2,2,2,2,2,2,2,2,2,2,2,2,2,2,2,2,2,2,2,2,2,2,2,2,2,2,2,2,2,
4),(-2.59347629365865,-2.58829257532513,-2.5411668967311,-2.51687818982104,
-2.50473142931873,-2.49785808943214,-2.49591737153289,-2.49490285462753,
-2.49383144840807,-2.49248355938424,-2.48986143190541,-2.47381247037154,
-2.46857792372863,-2.42101660746502,-2.40445238062561,-2.39414115779919,
-2.39089233110921,-2.38881892057753,-2.38687814957512,-2.3843368443699,
-2.38004159228423,-2.34490982704621,-2.29594431707583,-2.28624551428981,
-2.28407421432403,-2.28283987477601,-2.28176592354043,-2.28038695137753,
-2.27816588351489,-2.26581830620826,-2.26271188533856,-2.2554980111405,
-2.2143647193356,-2.18429814564924,-2.17987187928093,-2.17754187380324,
-2.17562996445238,-2.17341113183488,-2.16960586932928,-2.15480566428064,
-2.14257500429753,-2.10708124210635,-2.08472118800863,-2.07436930278858,
-2.0721546848398,-2.07091085958896,-2.06983819716764,-2.06847323943045,
-2.06577120476464,-2.04752376693149,-2.02951962955377,-1.99678709087343,
-1.97428208502551,-1.96863575959022,-1.96606571148314,-1.96412733601595,
-1.96230008081796,-1.95975637932984,-1.95310462516989,-1.89738998985074,
-1.87326204029726,-1.86242060551688,-1.86017539939669,-1.85892482506506,
-1.85785279594466,-1.85649693031458,-1.85435216700402,-1.84333052050339,
-1.7920312423049,-1.76336881456514,-1.75694036291911,-1.75423240096493,
-1.7522707046935,-1.75047772064283,-1.74761138835131,-1.7407194677468,-1.68772908512975,
-1.66175608240713,-1.65043163279768,-1.64815799909465,-1.64690125659645,
-1.64582982839145,-1.6444822262148,-1.64186158218782,-1.6258376692416,-1.62043556344291,
-1.60593574777678,-1.57304126179432,-1.55028558881354,-1.54460521787163,
-1.54202881306141,-1.54008935023846,-1.53826378903245,-1.53572680233329,
-1.52911838860071,-1.4729707930136,-1.44912251428612,-1.43835641248185,
-1.43611567424345,-1.43486602144414,-1.43379381485167,-1.43243648266648,
-1.42977082786721,-1.41258483359625,-1.36250940842122,-1.34495460388798,
-1.3342008367151,-1.33090191892753,-1.32881733320829,-1.32688051001754,
-1.32432142927179,-1.31873513605441,-1.31131206952259,-1.2927112038443,
-1.25986769515979),.UNSPECIFIED.);
#742=B_SPLINE_CURVE_WITH_KNOTS('',3,(#68406,#68407,#68408,#68409,#68410,
#68411,#68412,#68413,#68414,#68415,#68416,#68417,#68418,#68419),
 .UNSPECIFIED.,.F.,.F.,(4,2,2,2,2,2,4),(-0.0749178273173223,-0.0723413266242414,
-0.0418124322290516,-0.00539432297196826,-0.00193487110848845,-0.000864100279469971,
-0.000629065621366007),.UNSPECIFIED.);
#743=B_SPLINE_CURVE_WITH_KNOTS('',3,(#68420,#68421,#68422,#68423,#68424,
#68425,#68426,#68427,#68428,#68429,#68430,#68431,#68432,#68433,#68434,#68435,
#68436,#68437,#68438,#68439,#68440,#68441,#68442,#68443,#68444,#68445,#68446,
#68447,#68448,#68449,#68450,#68451,#68452,#68453,#68454,#68455,#68456,#68457,
#68458,#68459,#68460,#68461,#68462,#68463,#68464,#68465,#68466,#68467,#68468,
#68469,#68470,#68471,#68472,#68473,#68474,#68475,#68476,#68477,#68478,#68479,
#68480,#68481,#68482,#68483,#68484,#68485,#68486,#68487,#68488,#68489,#68490,
#68491,#68492,#68493,#68494,#68495,#68496,#68497,#68498,#68499,#68500,#68501,
#68502,#68503,#68504,#68505,#68506,#68507,#68508,#68509,#68510,#68511,#68512,
#68513,#68514,#68515,#68516,#68517,#68518,#68519,#68520,#68521,#68522,#68523,
#68524,#68525,#68526,#68527,#68528,#68529,#68530,#68531,#68532,#68533,#68534,
#68535,#68536,#68537,#68538,#68539,#68540,#68541,#68542,#68543,#68544,#68545,
#68546,#68547,#68548,#68549,#68550,#68551,#68552,#68553,#68554,#68555,#68556,
#68557,#68558,#68559,#68560,#68561,#68562,#68563,#68564,#68565,#68566,#68567,
#68568,#68569,#68570,#68571,#68572,#68573,#68574,#68575,#68576,#68577,#68578,
#68579,#68580,#68581,#68582,#68583,#68584,#68585,#68586,#68587,#68588,#68589,
#68590,#68591,#68592,#68593,#68594,#68595,#68596,#68597,#68598,#68599,#68600),
 .UNSPECIFIED.,.F.,.F.,(4,3,3,3,3,3,3,3,3,3,3,3,3,3,3,3,3,3,3,3,3,3,3,3,
3,3,3,3,3,3,3,3,3,3,3,3,3,3,3,3,3,3,3,3,3,3,3,3,3,3,3,3,3,3,3,3,3,3,3,3,
4),(145.822598481187,145.830121694434,145.93351643147,146.036757713572,
146.139877678952,146.242932247149,146.345955455495,146.448981298155,146.552114064922,
146.65530315632,146.758675149691,146.828958144396,146.932352881429,147.035594163529,
147.138714128907,147.2417686971,147.344791905443,147.4478177481,147.550950514863,
147.654139606257,147.757511599624,147.827794594357,147.931189331481,148.034430613672,
148.137550579141,148.240605147425,148.343628355859,148.446654198607,148.54978696546,
148.652976056944,148.756348050398,148.826631044319,148.930025781262,149.033267063272,
149.136387028561,149.239441596667,149.342464804923,149.445490647494,149.548623414173,
149.651812505485,149.755184498771,149.825467494281,149.928862231266,150.032103513316,
150.135223478642,150.238278046784,150.341301255073,150.444327097677,150.547459864385,
150.650648955725,150.754020949036,150.824303944243,150.927703487106,151.031158731356,
151.134277037909,151.237328088427,151.340345921593,151.444095801472,151.547200194451,
151.651272817779,151.755345441108),.UNSPECIFIED.);
#744=B_SPLINE_CURVE_WITH_KNOTS('',3,(#68602,#68603,#68604,#68605,#68606,
#68607,#68608,#68609,#68610,#68611,#68612,#68613,#68614,#68615,#68616,#68617,
#68618,#68619,#68620,#68621,#68622,#68623,#68624,#68625,#68626,#68627,#68628,
#68629,#68630,#68631,#68632,#68633,#68634,#68635,#68636,#68637,#68638,#68639,
#68640,#68641,#68642,#68643,#68644,#68645,#68646,#68647,#68648,#68649,#68650,
#68651,#68652,#68653,#68654,#68655,#68656,#68657,#68658,#68659,#68660,#68661,
#68662,#68663,#68664,#68665,#68666,#68667,#68668,#68669,#68670,#68671,#68672,
#68673,#68674,#68675,#68676,#68677,#68678,#68679,#68680,#68681,#68682,#68683,
#68684,#68685,#68686,#68687,#68688,#68689,#68690,#68691,#68692,#68693,#68694,
#68695,#68696,#68697,#68698,#68699,#68700,#68701,#68702,#68703,#68704,#68705,
#68706,#68707,#68708,#68709,#68710,#68711,#68712,#68713,#68714,#68715,#68716,
#68717,#68718,#68719,#68720,#68721,#68722,#68723,#68724,#68725,#68726,#68727,
#68728,#68729,#68730,#68731,#68732,#68733,#68734,#68735,#68736,#68737,#68738,
#68739,#68740,#68741,#68742,#68743,#68744,#68745,#68746,#68747,#68748,#68749,
#68750,#68751,#68752,#68753,#68754,#68755,#68756,#68757,#68758,#68759,#68760,
#68761,#68762,#68763,#68764,#68765,#68766,#68767,#68768,#68769,#68770,#68771,
#68772,#68773,#68774,#68775,#68776,#68777,#68778,#68779,#68780,#68781,#68782,
#68783,#68784,#68785,#68786,#68787,#68788,#68789,#68790,#68791,#68792,#68793,
#68794,#68795,#68796,#68797,#68798,#68799,#68800,#68801,#68802,#68803,#68804,
#68805,#68806,#68807,#68808,#68809,#68810,#68811,#68812,#68813,#68814,#68815,
#68816,#68817,#68818,#68819,#68820,#68821,#68822,#68823,#68824,#68825,#68826,
#68827),.UNSPECIFIED.,.F.,.F.,(4,2,2,2,2,2,2,2,2,2,2,2,2,2,2,2,2,2,2,2,
2,2,2,2,2,2,2,2,2,2,2,2,2,2,2,2,2,2,2,2,2,2,2,2,2,2,2,2,2,2,2,2,2,2,2,2,
2,2,2,2,2,2,2,2,2,2,2,2,2,2,2,2,2,2,2,2,2,2,2,2,2,2,2,2,2,2,2,2,2,2,2,2,
2,2,2,2,2,2,2,2,2,2,2,2,2,2,2,2,2,2,2,2,4),(-1.25986769515979,-1.2499844263308,
-1.2273577862635,-1.22450577490825,-1.22312919393204,-1.22205539983242,
-1.22081932328019,-1.21864036701087,-1.20883170496701,-1.15992913113595,
-1.12481181987302,-1.12051636491675,-1.11797495911435,-1.11603411154155,
-1.11396061854871,-1.11071166006578,-1.10039991255488,-1.08383704907641,
-1.05097559989016,-1.03714819275762,-1.03049858177144,-1.01502580013971,
-1.01242885687368,-1.01108642443104,-1.01001538880904,-1.00875478599536,
-1.00646309891425,-0.994817037352779,-0.967552171293446,-0.947368838057844,
-0.912862935943923,-0.908576485430226,-0.906037714206087,-0.904097325737947,
-0.902022815774536,-0.89876911199953,-0.888415649495207,-0.871760344990376,
-0.838822650589742,-0.820097325676813,-0.803187318670966,-0.800532350845072,
-0.79917744626026,-0.798105594584209,-0.796854563336167,-0.794606865326288,
-0.783721648218932,-0.759426221407249,-0.703933009258047,-0.69725755512765,
-0.694710329946686,-0.692882274966,-0.690944640687363,-0.688378266025517,
-0.682750918500276,-0.675258439804106,-0.656402509725772,-0.626239603600697,
-0.603910453728246,-0.590918431140894,-0.588663906675867,-0.587274966899738,
-0.586200150638521,-0.584972544910109,-0.582831270663668,-0.57355424355626,
-0.554763343083938,-0.545913352488733,-0.492210670271743,-0.485374614518985,
-0.482517793901791,-0.480726769064398,-0.478764004306589,-0.476048652516343,
-0.469574475530155,-0.440526057182572,-0.394674488142699,-0.379152289898522,
-0.376553533538344,-0.375210828710214,-0.374139928436181,-0.372879895432954,
-0.37059029811673,-0.359258417209125,-0.333150177798527,-0.281816442239883,
-0.273829151212125,-0.270784101753617,-0.268957978537776,-0.267019676727467,
-0.264447801193517,-0.259241715375701,-0.252198209225489,-0.234953887526279,
-0.197957856253062,-0.167653358059792,-0.164740323769206,-0.163352090118205,
-0.16227743845337,-0.161049593689972,-0.159757697637198,-0.15511185568413,
-0.128865267669617,-0.106990977580988,-0.105569210849635,-0.0651104303029907,
-0.0603738338460286,-0.0579480560258702,-0.056029046889496,-0.0538783718243573,
-0.0516516615518185,-0.0483298236007792,-0.000628984974797087),
 .UNSPECIFIED.);
#745=B_SPLINE_CURVE_WITH_KNOTS('',3,(#68828,#68829,#68830,#68831,#68832,
#68833,#68834,#68835,#68836,#68837,#68838,#68839,#68840,#68841,#68842,#68843,
#68844,#68845,#68846,#68847),.UNSPECIFIED.,.F.,.F.,(4,2,2,2,2,2,2,2,2,4),
(-2.6677982910831,-2.62484284417815,-2.62190879437548,-2.62022600193997,
-2.61872103544168,-2.61762940481273,-2.61660206215556,-2.6148524262143,
-2.61007806701873,-2.5936683297307),.UNSPECIFIED.);
#746=B_SPLINE_CURVE_WITH_KNOTS('',3,(#68852,#68853,#68854,#68855,#68856,
#68857,#68858,#68859,#68860,#68861,#68862,#68863,#68864,#68865,#68866,#68867,
#68868,#68869,#68870,#68871,#68872,#68873,#68874,#68875,#68876,#68877,#68878,
#68879,#68880,#68881,#68882,#68883,#68884,#68885,#68886,#68887,#68888,#68889,
#68890,#68891,#68892,#68893,#68894,#68895,#68896,#68897,#68898,#68899,#68900,
#68901,#68902,#68903,#68904,#68905,#68906,#68907,#68908,#68909,#68910,#68911,
#68912,#68913,#68914,#68915,#68916,#68917,#68918,#68919,#68920,#68921,#68922,
#68923,#68924,#68925,#68926,#68927,#68928,#68929,#68930,#68931,#68932,#68933,
#68934,#68935,#68936,#68937,#68938,#68939,#68940,#68941,#68942,#68943,#68944,
#68945,#68946,#68947,#68948,#68949,#68950,#68951,#68952,#68953,#68954,#68955,
#68956,#68957,#68958,#68959,#68960,#68961,#68962,#68963,#68964,#68965,#68966,
#68967,#68968,#68969,#68970,#68971,#68972,#68973,#68974,#68975,#68976,#68977,
#68978,#68979,#68980,#68981,#68982,#68983,#68984,#68985,#68986,#68987,#68988,
#68989,#68990,#68991,#68992,#68993,#68994,#68995,#68996,#68997,#68998,#68999,
#69000,#69001,#69002,#69003,#69004,#69005,#69006,#69007,#69008,#69009,#69010,
#69011,#69012,#69013,#69014,#69015,#69016,#69017,#69018,#69019,#69020,#69021,
#69022,#69023,#69024,#69025,#69026,#69027,#69028,#69029,#69030,#69031,#69032,
#69033,#69034,#69035,#69036,#69037,#69038,#69039,#69040,#69041,#69042,#69043,
#69044,#69045,#69046,#69047,#69048,#69049,#69050,#69051,#69052,#69053,#69054,
#69055,#69056,#69057,#69058,#69059,#69060,#69061,#69062,#69063,#69064,#69065,
#69066,#69067,#69068,#69069,#69070,#69071,#69072,#69073,#69074,#69075,#69076,
#69077,#69078,#69079,#69080,#69081,#69082,#69083,#69084,#69085,#69086,#69087,
#69088,#69089,#69090,#69091,#69092,#69093,#69094,#69095,#69096,#69097,#69098,
#69099,#69100,#69101,#69102,#69103,#69104,#69105,#69106,#69107,#69108,#69109,
#69110,#69111,#69112,#69113,#69114,#69115,#69116,#69117,#69118,#69119,#69120,
#69121,#69122,#69123,#69124,#69125),.UNSPECIFIED.,.F.,.F.,(4,2,2,2,2,2,
2,2,2,2,2,2,2,2,2,2,2,2,2,2,2,2,2,2,2,2,2,2,2,2,2,2,2,2,2,2,2,2,2,2,2,2,
2,2,2,2,2,2,2,2,2,2,2,2,2,2,2,2,2,2,2,2,2,2,2,2,2,2,2,2,2,2,2,2,2,2,2,2,
2,2,2,2,2,2,2,2,2,2,2,2,2,2,2,2,2,2,2,2,2,2,2,2,2,2,2,2,2,2,2,2,2,2,2,2,
2,2,2,2,2,2,2,2,2,2,2,2,2,2,2,2,2,2,2,2,2,2,4),(-1.40862414609624,-1.39318980279119,
-1.38284072661476,-1.37958737276298,-1.37751284603091,-1.37557227418975,
-1.37303302268065,-1.36874525537374,-1.33415944586128,-1.2781862454669,
-1.27391184913531,-1.27224005010757,-1.27122788636052,-1.27012540359843,
-1.26856027607177,-1.2646472311334,-1.24543237740231,-1.189051015541,-1.17220367699145,
-1.16858648625196,-1.1662220751037,-1.1643080269843,-1.16211558550351,-1.15832879058625,
-1.14208004095366,-1.08459839210323,-1.07962518793354,-1.06363760215019,
-1.06101890048426,-1.05967166679635,-1.05860019941163,-1.05734303160051,
-1.05506765324818,-1.04371503635272,-1.01762985177148,-0.964752180156942,
-0.957848408238544,-0.954980018513344,-0.95318658397866,-0.951225072691281,
-0.948518600603874,-0.942099509999168,-0.913520898721511,-0.862318476563556,
-0.851156478542139,-0.849003060786239,-0.847644536526994,-0.846572282368348,
-0.845323607248431,-0.843087178903938,-0.832390627380297,-0.808794013748438,
-0.75222100751256,-0.745655083270969,-0.743124936486027,-0.741301236761814,
-0.73936092215405,-0.736778539925796,-0.731065044743599,-0.708064530032574,
-0.67504301687471,-0.653990204817018,-0.647228276238945,-0.638780487972627,
-0.636628936585396,-0.635386248131689,-0.634313429629788,-0.632946801850073,
-0.630144870928438,-0.596426883720288,-0.54028254859855,-0.533672456392464,
-0.531135432182919,-0.529310043610141,-0.527370948020244,-0.524795337208315,
-0.519117959943133,-0.496384070865972,-0.463534763653935,-0.427913975639064,
-0.425051291782673,-0.423672766840067,-0.422598961154527,-0.421364568781365,
-0.419192637218565,-0.409482528108991,-0.360507265752088,-0.325369848208395,
-0.321074835958497,-0.318533798237304,-0.316593292897703,-0.314520224798732,
-0.311272055836028,-0.300963857377367,-0.28440768653318,-0.233328469855719,
-0.231093888984576,-0.215559530390286,-0.212981629890186,-0.211658069355316,
-0.210638095905596,-0.210630093278843,-0.210622259266652,-0.210614583458265,
-0.210607056158067,-0.210599668548909,-0.210592412317678,-0.210585279938524,
-0.210578264423103,-0.210571359038716,-0.210564557512432,-0.210557854162641,
-0.210551243629364,-0.210544720702707,-0.21053828046371,-0.210531918507408,
-0.210525630626156,-0.21051941260701,-0.210513260713285,-0.210507171285705,
-0.21050114086118,-0.210495166127197,-0.210489243937745,-0.210483371400245,
-0.210477545698568,-0.209214406034747,-0.206826847606485,-0.19326725644468,
-0.157092503551496,-0.113387632942077,-0.109098752214622,-0.10655954168276,
-0.104619394012564,-0.10254570114519,-0.0992944491784891,-0.0889586946482435,
-0.0749178273173223),.UNSPECIFIED.);
#747=B_SPLINE_CURVE_WITH_KNOTS('',3,(#69126,#69127,#69128,#69129,#69130,
#69131,#69132,#69133,#69134,#69135,#69136,#69137,#69138,#69139,#69140,#69141,
#69142,#69143,#69144,#69145,#69146,#69147,#69148,#69149,#69150,#69151,#69152,
#69153,#69154,#69155,#69156,#69157,#69158,#69159,#69160,#69161,#69162,#69163,
#69164,#69165,#69166,#69167,#69168,#69169,#69170,#69171,#69172,#69173,#69174,
#69175,#69176,#69177,#69178,#69179,#69180,#69181,#69182,#69183,#69184,#69185,
#69186,#69187,#69188,#69189,#69190,#69191,#69192,#69193,#69194,#69195,#69196,
#69197,#69198,#69199,#69200,#69201,#69202,#69203,#69204,#69205,#69206,#69207,
#69208,#69209,#69210,#69211,#69212,#69213,#69214,#69215,#69216,#69217,#69218,
#69219,#69220,#69221,#69222,#69223,#69224,#69225,#69226,#69227,#69228,#69229,
#69230,#69231,#69232,#69233,#69234,#69235,#69236,#69237,#69238,#69239,#69240,
#69241,#69242,#69243,#69244,#69245,#69246,#69247,#69248,#69249,#69250,#69251,
#69252,#69253,#69254,#69255,#69256,#69257,#69258,#69259,#69260,#69261,#69262,
#69263,#69264,#69265,#69266,#69267,#69268,#69269,#69270,#69271,#69272,#69273,
#69274,#69275,#69276,#69277,#69278,#69279,#69280,#69281,#69282,#69283,#69284,
#69285,#69286,#69287,#69288,#69289,#69290,#69291,#69292,#69293,#69294,#69295,
#69296,#69297,#69298,#69299,#69300,#69301,#69302,#69303,#69304,#69305,#69306,
#69307,#69308,#69309,#69310,#69311,#69312,#69313,#69314,#69315,#69316,#69317,
#69318,#69319,#69320,#69321,#69322,#69323,#69324,#69325,#69326,#69327,#69328,
#69329,#69330,#69331,#69332,#69333,#69334,#69335,#69336,#69337,#69338,#69339,
#69340,#69341,#69342,#69343,#69344,#69345,#69346,#69347,#69348,#69349,#69350,
#69351,#69352,#69353,#69354,#69355,#69356,#69357),.UNSPECIFIED.,.F.,.F.,
(4,2,2,2,2,2,2,2,2,2,2,2,2,2,2,2,2,2,2,2,2,2,2,2,2,2,2,2,2,2,2,2,2,2,2,
2,2,2,2,2,2,2,2,2,2,2,2,2,2,2,2,2,2,2,2,2,2,2,2,2,2,2,2,2,2,2,2,2,2,2,2,
2,2,2,2,2,2,2,2,2,2,2,2,2,2,2,2,2,2,2,2,2,2,2,2,2,2,2,2,2,2,2,2,2,2,2,2,
2,2,2,2,2,2,2,2,4),(-2.5936683297307,-2.5726207840679,-2.55119822559827,
-2.52286135770751,-2.51638838092519,-2.51426413649379,-2.51218418040178,
-2.51024532309731,-2.50771804735601,-2.50347214253205,-2.47125311799585,
-2.43576565912732,-2.41832802532113,-2.40950864041021,-2.40740843522256,
-2.4061801278211,-2.40510499243148,-2.40371601917802,-2.40080104535941,
-2.3706852886388,-2.31914736690955,-2.31048993812756,-2.30424070509671,
-2.30153110187088,-2.29956889863741,-2.29777592025381,-2.29491061704547,
-2.2880264542602,-2.23491463762945,-2.20901717245987,-2.19771130706315,
-2.19543851015384,-2.19418184086959,-2.19311023869051,-2.19176211668817,
-2.1891395762449,-2.1730887360403,-2.16783995619816,-2.15321513168035,-2.12031456163141,
-2.10374303951701,-2.09342781749038,-2.09017801912045,-2.08810405773785,
-2.08616281978226,-2.0836209733347,-2.0793249637779,-2.04420790571177,-1.99530255525716,
-1.98551591591854,-1.98333821708696,-1.98210228269514,-1.98102825171372,
-1.97965088664476,-1.97679561477164,-1.9538281481496,-1.95168520789728,
-1.91152613950497,-1.89283640251648,-1.88158938989891,-1.878236792081,-1.87614013048961,
-1.8742069566071,-1.87171694656131,-1.8675985967015,-1.84074921139561,-1.79877078660577,
-1.78196749243118,-1.77334179158195,-1.77124909985302,-1.77003193385426,
-1.76895464362035,-1.76757038233075,-1.7652825972158,-1.75163464434942,
-1.74988584604178,-1.70251515946709,-1.67153888852473,-1.66708667104672,
-1.66475093468465,-1.66283834912034,-1.66062326542956,-1.65683551969551,
-1.64224021250126,-1.6299740707683,-1.58956098626714,-1.57070633717263,
-1.56140707116998,-1.55926368223693,-1.55803533939617,-1.55696019326658,
-1.55557123290499,-1.55265638065077,-1.52381683594311,-1.48570476804185,
-1.46817820092768,-1.45743650849027,-1.45413866485049,-1.45205414839308,
-1.4501169686029,-1.44760031308069,-1.44339085464906,-1.41291513139376,
-1.36768694294417,-1.35579379322469,-1.35125847821227,-1.34794990407903,
-1.34648734813586,-1.34540259097681,-1.34421364338769,-1.3422475989548,
-1.33584217266315,-1.33428618716082,-1.31969892252657,-1.26065445785916,
-1.25983890058673),.UNSPECIFIED.);
#748=B_SPLINE_CURVE_WITH_KNOTS('',3,(#69363,#69364,#69365,#69366,#69367,
#69368,#69369,#69370),.UNSPECIFIED.,.F.,.F.,(4,2,2,4),(-0.0748543400333247,
-0.0730685011140681,-0.0491237947608074,-0.000629479192835824),
 .UNSPECIFIED.);
#749=B_SPLINE_CURVE_WITH_KNOTS('',3,(#69371,#69372,#69373,#69374,#69375,
#69376,#69377,#69378,#69379,#69380,#69381,#69382,#69383,#69384,#69385,#69386,
#69387,#69388,#69389,#69390,#69391,#69392,#69393,#69394,#69395,#69396,#69397,
#69398,#69399,#69400,#69401,#69402,#69403,#69404,#69405,#69406,#69407,#69408,
#69409,#69410,#69411,#69412,#69413,#69414,#69415,#69416,#69417,#69418,#69419,
#69420,#69421,#69422,#69423,#69424,#69425,#69426,#69427,#69428,#69429,#69430,
#69431,#69432,#69433,#69434,#69435,#69436,#69437,#69438,#69439,#69440,#69441,
#69442,#69443,#69444,#69445,#69446,#69447,#69448,#69449,#69450,#69451,#69452,
#69453,#69454,#69455,#69456,#69457,#69458,#69459,#69460,#69461,#69462,#69463,
#69464,#69465,#69466,#69467,#69468,#69469,#69470,#69471,#69472,#69473,#69474,
#69475,#69476,#69477,#69478,#69479,#69480,#69481,#69482,#69483,#69484,#69485,
#69486,#69487,#69488,#69489,#69490,#69491,#69492,#69493,#69494,#69495,#69496,
#69497,#69498,#69499,#69500,#69501,#69502,#69503,#69504,#69505,#69506,#69507,
#69508,#69509,#69510,#69511,#69512,#69513,#69514,#69515,#69516,#69517,#69518,
#69519,#69520,#69521,#69522,#69523,#69524,#69525,#69526,#69527,#69528,#69529,
#69530,#69531,#69532,#69533,#69534,#69535,#69536,#69537,#69538,#69539,#69540,
#69541,#69542,#69543,#69544,#69545,#69546,#69547,#69548,#69549,#69550,#69551,
#69552,#69553,#69554,#69555,#69556,#69557,#69558,#69559,#69560,#69561,#69562,
#69563,#69564,#69565,#69566,#69567,#69568,#69569,#69570,#69571,#69572,#69573,
#69574,#69575,#69576,#69577,#69578,#69579,#69580,#69581,#69582,#69583,#69584,
#69585,#69586,#69587,#69588,#69589,#69590,#69591,#69592,#69593,#69594,#69595,
#69596,#69597,#69598,#69599,#69600,#69601,#69602,#69603,#69604,#69605,#69606,
#69607,#69608,#69609,#69610,#69611,#69612,#69613,#69614,#69615,#69616,#69617,
#69618,#69619,#69620,#69621,#69622,#69623,#69624,#69625,#69626,#69627,#69628),
 .UNSPECIFIED.,.F.,.F.,(4,2,2,2,2,2,2,2,2,2,2,2,2,2,2,2,2,2,2,2,2,2,2,2,
2,2,2,2,2,2,2,2,2,2,2,2,2,2,2,2,2,2,2,2,2,2,2,2,2,2,2,2,2,2,2,2,2,2,2,2,
2,2,2,2,2,2,2,2,2,2,2,2,2,2,2,2,2,2,2,2,2,2,2,2,2,2,2,2,2,2,2,2,2,2,2,2,
2,2,2,2,2,2,2,2,2,2,2,2,2,2,2,2,2,2,2,2,2,2,2,2,2,2,2,2,2,2,2,2,4),(-2.66814368829348,
-2.66034873118431,-2.65505152358494,-2.65260779199081,-2.65072566522708,
-2.6488846910573,-2.64705802280244,-2.64451726183137,-2.63932533848064,
-2.62681330898061,-2.57513659029226,-2.55629150625919,-2.54699526628027,
-2.54485209086409,-2.54362379238626,-2.54254863419885,-2.54115959109167,
-2.53824432801602,-2.50854367015596,-2.45808754405171,-2.44859722597837,
-2.44398932066425,-2.44020970600377,-2.43803870623047,-2.43802300969667,
-2.4380067605024,-2.43798993855578,-2.43797252300731,-2.43795449224214,
-2.43793582387495,-2.4379164947004,-2.43789648064213,-2.43787575678477,
-2.4378542973178,-2.43783207551628,-2.43780906301748,-2.43778902406746,
-2.4377656706735,-2.43773846067708,-2.43770676597262,-2.43766986014221,
-2.43762690482853,-2.4375726852995,-2.43563170291138,-2.43308934965835,
-2.42879059675919,-2.39366442341326,-2.34469891665934,-2.33499836395926,
-2.33282690447066,-2.33159251024439,-2.33051853457682,-2.32913956130739,
-2.32627516729251,-2.29031752177012,-2.2575466302749,-2.23498252385049,
-2.22932813927916,-2.22675657538432,-2.22481793266635,-2.22299106930673,
-2.22044894667414,-2.21380749423047,-2.15799208910578,-2.13392861942916,
-2.12310446786992,-2.12086027325997,-2.1196099025175,-2.11853782608796,
-2.11718161605693,-2.1150357747995,-2.10399726717983,-2.05277424947031,
-2.02406100664172,-2.0176264316783,-2.01491739871002,-2.01295547388808,
-2.01116265737428,-2.00829741164116,-2.00141234454558,-1.94832934653784,
-1.92241930829777,-1.91111079398823,-1.90883803777882,-1.90758146809275,
-1.90650999765976,-1.90516210101186,-1.90254017435152,-1.8864959682302,
-1.88120554232293,-1.86661833145533,-1.8337220866743,-1.81715303187371,
-1.80683926115751,-1.80358987508024,-1.80151616601908,-1.79957515665534,
-1.79703359858572,-1.79273805190484,-1.75762153288418,-1.70871089440112,
-1.69893858239314,-1.6967620416682,-1.69552645190864,-1.69445252034459,
-1.69307502126333,-1.69021857225249,-1.66741781584811,-1.61179980388429,
-1.59578596449105,-1.59201598172407,-1.58982721629583,-1.58791275959955,
-1.58554317036637,-1.58190933911534,-1.56481024540013,-1.55674001414502,
-1.52192473962697,-1.49787209418288,-1.48705111597682,-1.48480720636253,
-1.48355694212671,-1.48248492478154,-1.48112874813835,-1.47846810954277,
-1.46141221384331,-1.44279783998196,-1.40983725064088,-1.40862414609624),
 .UNSPECIFIED.);
#750=B_SPLINE_CURVE_WITH_KNOTS('',3,(#69630,#69631,#69632,#69633,#69634,
#69635,#69636,#69637,#69638,#69639,#69640,#69641,#69642,#69643,#69644,#69645,
#69646,#69647,#69648,#69649,#69650,#69651,#69652,#69653,#69654,#69655,#69656,
#69657,#69658,#69659,#69660,#69661,#69662,#69663,#69664,#69665,#69666,#69667,
#69668,#69669,#69670,#69671,#69672,#69673,#69674,#69675,#69676,#69677,#69678,
#69679,#69680,#69681,#69682,#69683,#69684,#69685,#69686,#69687,#69688,#69689,
#69690,#69691,#69692,#69693,#69694,#69695,#69696,#69697,#69698,#69699,#69700,
#69701,#69702,#69703,#69704,#69705,#69706,#69707,#69708,#69709,#69710,#69711,
#69712,#69713,#69714,#69715,#69716,#69717,#69718,#69719,#69720,#69721,#69722,
#69723,#69724,#69725,#69726,#69727,#69728,#69729,#69730,#69731,#69732,#69733,
#69734,#69735,#69736,#69737,#69738,#69739,#69740,#69741,#69742,#69743,#69744,
#69745,#69746,#69747,#69748,#69749,#69750,#69751,#69752,#69753,#69754,#69755,
#69756,#69757,#69758,#69759,#69760,#69761,#69762,#69763,#69764,#69765,#69766,
#69767,#69768,#69769,#69770,#69771,#69772,#69773,#69774,#69775,#69776,#69777,
#69778,#69779,#69780,#69781,#69782,#69783,#69784,#69785,#69786,#69787,#69788,
#69789,#69790,#69791,#69792,#69793,#69794,#69795,#69796,#69797,#69798,#69799,
#69800,#69801,#69802,#69803,#69804,#69805,#69806,#69807,#69808,#69809,#69810,
#69811,#69812,#69813,#69814,#69815,#69816,#69817,#69818,#69819,#69820,#69821,
#69822,#69823,#69824,#69825,#69826,#69827,#69828,#69829,#69830,#69831,#69832,
#69833,#69834,#69835,#69836,#69837,#69838,#69839,#69840,#69841),
 .UNSPECIFIED.,.F.,.F.,(4,2,2,2,2,2,2,2,2,2,2,2,2,2,2,2,2,2,2,2,2,2,2,2,
2,2,2,2,2,2,2,2,2,2,2,2,2,2,2,2,2,2,2,2,2,2,2,2,2,2,2,2,2,2,2,2,2,2,2,2,
2,2,2,2,2,2,2,2,2,2,2,2,2,2,2,2,2,2,2,2,2,2,2,2,2,2,2,2,2,2,2,2,2,2,2,2,
2,2,2,2,2,2,2,2,2,4),(-1.25983890058673,-1.24634406344438,-1.24258219161815,
-1.24037324998251,-1.23846050074872,-1.23611765858758,-1.23163051026512,
-1.19926717360426,-1.15908299348593,-1.1541501744994,-1.13819946766059,
-1.13558278234653,-1.13423599916244,-1.13316458106479,-1.13190711265831,
-1.1296302780235,-1.1182515945149,-1.09206315122662,-1.03933492965326,-1.03242027292118,
-1.02955012835499,-1.02775640087641,-1.02579521475537,-1.02309037344317,
-1.01668073355414,-0.988180701441149,-0.937248744330339,-0.925763770623649,
-0.923591050901342,-0.922226669260455,-0.921153966790587,-0.919909539851915,
-0.917692476034015,-0.907304808266461,-0.884817221689897,-0.826488685982098,
-0.820131081486876,-0.817635177981923,-0.815820450706279,-0.813874971674538,
-0.811260203321051,-0.8053673892928,-0.78100871753366,-0.730336180278094,
-0.714124144264271,-0.711496163020898,-0.710147000641374,-0.709075492226207,
-0.707820004520276,-0.705552050381173,-0.694325812729196,-0.668733325368552,
-0.61515331894606,-0.608305517771778,-0.605446487862613,-0.603654862354507,
-0.601692072007581,-0.598977849116755,-0.592511919936247,-0.538387101565756,
-0.502385066625971,-0.499523482558151,-0.498145071609489,-0.497071159822568,
-0.495836425627053,-0.493663367892962,-0.483939608367895,-0.434968805203786,
-0.399816974208812,-0.395528974833991,-0.39298980903015,-0.391049420450672,
-0.388975203055071,-0.385722570313168,-0.375377700659135,-0.358741168315753,
-0.325819822418563,-0.307757445673727,-0.290182369777355,-0.287503244684659,
-0.28614321277118,-0.285071011863426,-0.283823823813925,-0.281593590316445,
-0.270992728538176,-0.247741175267763,-0.192010060381105,-0.18452885394621,
-0.181563540173496,-0.179752471417974,-0.177922125735423,-0.175416890437485,
-0.170092083543928,-0.163020954964638,-0.145679755924338,-0.097270332702688,
-0.0924434285828069,-0.0779766547156677,-0.075650015844025,-0.0742546067190068,
-0.0731762444961421,-0.0719663774955741,-0.0699052135922942,-0.0616645216555707,
-0.0459685411644556,-0.000629550022902194),.UNSPECIFIED.);
#751=B_SPLINE_CURVE_WITH_KNOTS('',3,(#69842,#69843,#69844,#69845,#69846,
#69847,#69848,#69849,#69850,#69851,#69852,#69853,#69854,#69855,#69856,#69857,
#69858,#69859,#69860,#69861,#69862,#69863),.UNSPECIFIED.,.F.,.F.,(4,2,2,
2,2,2,2,2,2,2,4),(-2.667696362868,-2.64236919542473,-2.63924210061828,-2.63709594523076,
-2.63529507404303,-2.63338105697752,-2.63101180962497,-2.62737812380157,
-2.61027214598184,-2.59808114560931,-2.59327317464725),.UNSPECIFIED.);
#752=B_SPLINE_CURVE_WITH_KNOTS('',3,(#69868,#69869,#69870,#69871,#69872,
#69873,#69874,#69875,#69876,#69877,#69878,#69879,#69880,#69881,#69882,#69883,
#69884,#69885,#69886,#69887,#69888,#69889,#69890,#69891,#69892,#69893,#69894,
#69895,#69896,#69897,#69898,#69899,#69900,#69901,#69902,#69903,#69904,#69905,
#69906,#69907,#69908,#69909,#69910,#69911,#69912,#69913,#69914,#69915,#69916,
#69917,#69918,#69919,#69920,#69921,#69922,#69923,#69924,#69925,#69926,#69927,
#69928,#69929,#69930,#69931,#69932,#69933,#69934,#69935,#69936,#69937,#69938,
#69939,#69940,#69941,#69942,#69943,#69944,#69945,#69946,#69947,#69948,#69949,
#69950,#69951,#69952,#69953,#69954,#69955,#69956,#69957,#69958,#69959,#69960,
#69961,#69962,#69963,#69964,#69965,#69966,#69967,#69968,#69969,#69970,#69971,
#69972,#69973,#69974,#69975,#69976,#69977,#69978,#69979,#69980,#69981,#69982,
#69983,#69984,#69985,#69986,#69987,#69988,#69989,#69990,#69991,#69992,#69993,
#69994,#69995,#69996,#69997,#69998,#69999,#70000,#70001,#70002,#70003,#70004,
#70005,#70006,#70007,#70008,#70009,#70010,#70011,#70012,#70013,#70014,#70015,
#70016,#70017,#70018,#70019,#70020,#70021,#70022,#70023,#70024,#70025,#70026,
#70027,#70028,#70029,#70030,#70031,#70032,#70033,#70034,#70035,#70036,#70037,
#70038,#70039,#70040,#70041,#70042,#70043,#70044,#70045,#70046,#70047,#70048,
#70049,#70050,#70051,#70052,#70053,#70054,#70055,#70056,#70057,#70058,#70059,
#70060,#70061,#70062,#70063,#70064,#70065,#70066,#70067,#70068,#70069,#70070,
#70071,#70072,#70073,#70074,#70075,#70076,#70077,#70078,#70079,#70080,#70081,
#70082,#70083,#70084,#70085,#70086,#70087,#70088,#70089,#70090,#70091,#70092,
#70093,#70094,#70095,#70096,#70097,#70098,#70099,#70100,#70101,#70102,#70103,
#70104,#70105,#70106,#70107,#70108,#70109),.UNSPECIFIED.,.F.,.F.,(4,2,2,
2,2,2,2,2,2,2,2,2,2,2,2,2,2,2,2,2,2,2,2,2,2,2,2,2,2,2,2,2,2,2,2,2,2,2,2,
2,2,2,2,2,2,2,2,2,2,2,2,2,2,2,2,2,2,2,2,2,2,2,2,2,2,2,2,2,2,2,2,2,2,2,2,
2,2,2,2,2,2,2,2,2,2,2,2,2,2,2,2,2,2,2,2,2,2,2,2,2,2,2,2,2,2,2,2,2,2,2,2,
2,2,2,2,2,2,2,2,2,4),(-1.40834652030694,-1.40119964678896,-1.3750453295523,
-1.36367482587345,-1.36139854842979,-1.36014122842095,-1.35906984371272,
-1.35772297797095,-1.35510576847566,-1.33914378880401,-1.33419979165065,
-1.32855380466372,-1.28159454650626,-1.28014905551357,-1.26110947023717,
-1.25734830242951,-1.25493954883956,-1.25302179779228,-1.25085960514823,
-1.24720980334545,-1.2327575183561,-1.18237043657965,-1.1527028321594,-1.1497883459888,
-1.14839958362139,-1.14732459775158,-1.14609645511031,-1.14395344114746,
-1.13465649989949,-1.11580505635895,-1.07535189164056,-1.06307322427455,
-1.04849344934274,-1.04470748206018,-1.04249303256104,-1.04058074806373,
-1.03824506925409,-1.03379200257817,-1.002756085599,-0.954779146164212,
-0.940189593244896,-0.93785721640681,-0.936459975086064,-0.935381181248489,
-0.934171927756229,-0.932114237676863,-0.923919063393083,-0.90835353979627,
-0.866772127234862,-0.854686082958407,-0.836943624112443,-0.833267940453417,
-0.830885427656707,-0.828969951331454,-0.826790253764856,-0.823061439572297,
-0.807603545846204,-0.755931244369677,-0.728679182947644,-0.725775379934821,
-0.724388660243346,-0.723313849021782,-0.722084330554783,-0.719935218297145,
-0.710554369962836,-0.661283712197524,-0.626052679490348,-0.621755690793678,
-0.619213822412307,-0.617272877714507,-0.615199529265458,-0.611951315626917,
-0.60164630011947,-0.585098401745746,-0.552249102173091,-0.539739318930592,
-0.516621656941801,-0.513764052151514,-0.512386448205456,-0.511312644072672,
-0.510077445504139,-0.507902165131855,-0.49814530336416,-0.449204353142808,
-0.414077528364177,-0.409781556887335,-0.407240121406575,-0.405299410053123,
-0.403226216624753,-0.399978049116185,-0.389671522433624,-0.373119621693654,
-0.34026903733369,-0.327235070420115,-0.318518706322198,-0.304213318370959,
-0.301892997747478,-0.300499430127896,-0.299421295226148,-0.298210346503724,
-0.296144370484358,-0.287845384120449,-0.271983674965682,-0.22595801836517,
-0.201643903831069,-0.197626207315011,-0.195166461523407,-0.193295990106968,
-0.191268163552431,-0.188078056392624,-0.184324499429698,-0.177192650513944,
-0.159636482061495,-0.109560650108114,-0.0924412901657382,-0.0897787049546927,
-0.0884222410408426,-0.087350360247461,-0.0861006799385381,-0.0838588658302869,
-0.0748543400333247),.UNSPECIFIED.);
#753=B_SPLINE_CURVE_WITH_KNOTS('',3,(#70110,#70111,#70112,#70113,#70114,
#70115,#70116,#70117,#70118,#70119,#70120,#70121,#70122,#70123,#70124,#70125,
#70126,#70127,#70128,#70129,#70130,#70131,#70132,#70133,#70134,#70135,#70136,
#70137,#70138,#70139,#70140,#70141,#70142,#70143,#70144,#70145,#70146,#70147,
#70148,#70149,#70150,#70151,#70152,#70153,#70154,#70155,#70156,#70157,#70158,
#70159,#70160,#70161,#70162,#70163,#70164,#70165,#70166,#70167,#70168,#70169,
#70170,#70171,#70172,#70173,#70174,#70175,#70176,#70177,#70178,#70179,#70180,
#70181,#70182,#70183,#70184,#70185,#70186,#70187,#70188,#70189,#70190,#70191,
#70192,#70193,#70194,#70195,#70196,#70197,#70198,#70199,#70200,#70201,#70202,
#70203,#70204,#70205,#70206,#70207,#70208,#70209,#70210,#70211,#70212,#70213,
#70214,#70215,#70216,#70217,#70218,#70219,#70220,#70221,#70222,#70223,#70224,
#70225,#70226,#70227,#70228,#70229,#70230,#70231,#70232,#70233,#70234,#70235,
#70236,#70237,#70238,#70239,#70240,#70241,#70242,#70243,#70244,#70245,#70246,
#70247,#70248,#70249,#70250,#70251,#70252,#70253,#70254,#70255,#70256,#70257,
#70258,#70259,#70260,#70261,#70262,#70263,#70264,#70265,#70266,#70267,#70268,
#70269,#70270,#70271,#70272,#70273,#70274,#70275,#70276,#70277,#70278,#70279,
#70280,#70281,#70282,#70283,#70284,#70285,#70286,#70287,#70288,#70289,#70290,
#70291,#70292,#70293,#70294,#70295,#70296,#70297,#70298,#70299,#70300,#70301,
#70302,#70303,#70304,#70305,#70306,#70307,#70308,#70309,#70310,#70311,#70312,
#70313,#70314,#70315,#70316,#70317,#70318,#70319,#70320,#70321,#70322,#70323,
#70324,#70325,#70326,#70327,#70328,#70329,#70330,#70331,#70332,#70333,#70334,
#70335,#70336,#70337,#70338,#70339),.UNSPECIFIED.,.F.,.F.,(4,2,2,2,2,2,
2,2,2,2,2,2,2,2,2,2,2,2,2,2,2,2,2,2,2,2,2,2,2,2,2,2,2,2,2,2,2,2,2,2,2,2,
2,2,2,2,2,2,2,2,2,2,2,2,2,2,2,2,2,2,2,2,2,2,2,2,2,2,2,2,2,2,2,2,2,2,2,2,
2,2,2,2,2,2,2,2,2,2,2,2,2,2,2,2,2,2,2,2,2,2,2,2,2,2,2,2,2,2,2,2,2,2,2,2,
4),(-2.59327317464725,-2.5704590027846,-2.54404918097376,-2.53261552028791,
-2.53033608522694,-2.5290782841031,-2.52800725378591,-2.52666180509699,
-2.52405019688048,-2.50827802161836,-2.50219760153401,-2.48282618273537,
-2.45493277432578,-2.43856538231164,-2.43177383929103,-2.42660779292877,
-2.42413937703768,-2.4222998924718,-2.42047511511372,-2.41793999218273,
-2.41134096218204,-2.35511961642112,-2.33133628620871,-2.32058892226935,
-2.31834972848019,-2.31710060479993,-2.31602864689801,-2.31467136584933,
-2.31252153835837,-2.30141357383613,-2.25015852191306,-2.22155602401871,
-2.21513527000744,-2.2124289049315,-2.21046776747491,-2.20867488257282,
-2.20580781280618,-2.19890947715483,-2.14603385775022,-2.11999207485746,
-2.10865099916055,-2.10637670979702,-2.10511996465956,-2.10404875247291,
-2.10270169977916,-2.10008294074918,-2.08408638148977,-2.07858665334349,
-2.06415914998794,-2.03127147490742,-2.0147079811946,-2.00439730764157,
-2.00114870346013,-1.99907544681252,-1.99713482819271,-1.99459373455749,
-1.99029886703047,-1.95517383607453,-1.90622460815131,-1.89651182976436,
-1.89433968318877,-1.89310521584231,-1.89203138021895,-1.89065285328871,
-1.88843307926109,-1.87610725052837,-1.8729791507541,-1.87277770786138,
-1.86591077771597,-1.8521781256169,-1.81929555402153,-1.80273984895054,
-1.79243249631211,-1.78918412564446,-1.78711082267907,-1.78517002347376,
-1.78262849535985,-1.77833244964047,-1.74313778478156,-1.69396685742474,
-1.68450731601472,-1.68235275394786,-1.68112210340309,-1.68004759568449,
-1.67866295841088,-1.67576945747559,-1.64973504199282,-1.61156794503932,
-1.58253999009771,-1.57814437560976,-1.57582080172747,-1.57390919438664,
-1.5716850692273,-1.5678568102575,-1.55279545393319,-1.50062697925078,-1.48178138712014,
-1.47248554193453,-1.47034264219521,-1.46911453147393,-1.46803955704983,
-1.46665077698046,-1.4637361564445,-1.43368995263626,-1.38234822370932,
-1.369008011865,-1.36545296099196,-1.36331180205574,-1.36139051569147,-1.35894717976743,
-1.3550726159874,-1.33399840580333,-1.2761823698615,-1.26122152598105,-1.2597871053314),
 .UNSPECIFIED.);
#754=B_SPLINE_CURVE_WITH_KNOTS('',3,(#70345,#70346,#70347,#70348),
 .UNSPECIFIED.,.F.,.F.,(4,4),(120.339865638913,120.689851223516),
 .UNSPECIFIED.);
#755=B_SPLINE_CURVE_WITH_KNOTS('',3,(#70349,#70350,#70351,#70352,#70353,
#70354,#70355,#70356,#70357,#70358,#70359,#70360,#70361,#70362,#70363,#70364,
#70365,#70366,#70367,#70368,#70369,#70370,#70371,#70372,#70373,#70374,#70375,
#70376,#70377,#70378,#70379,#70380,#70381,#70382,#70383,#70384,#70385,#70386,
#70387,#70388,#70389,#70390,#70391,#70392,#70393,#70394,#70395,#70396,#70397,
#70398,#70399,#70400,#70401,#70402,#70403,#70404,#70405,#70406,#70407,#70408,
#70409,#70410,#70411,#70412,#70413,#70414,#70415,#70416,#70417,#70418,#70419,
#70420,#70421,#70422,#70423,#70424,#70425,#70426,#70427,#70428,#70429,#70430,
#70431,#70432,#70433,#70434,#70435,#70436,#70437,#70438,#70439,#70440,#70441,
#70442,#70443,#70444,#70445,#70446,#70447,#70448,#70449,#70450,#70451,#70452,
#70453,#70454,#70455,#70456,#70457,#70458,#70459,#70460,#70461,#70462,#70463,
#70464,#70465,#70466,#70467,#70468,#70469,#70470,#70471,#70472,#70473,#70474,
#70475,#70476,#70477,#70478,#70479,#70480,#70481,#70482,#70483,#70484,#70485,
#70486,#70487,#70488,#70489,#70490,#70491,#70492,#70493,#70494,#70495,#70496,
#70497,#70498,#70499,#70500,#70501,#70502,#70503,#70504,#70505,#70506,#70507,
#70508,#70509,#70510,#70511,#70512,#70513,#70514,#70515,#70516,#70517,#70518,
#70519,#70520,#70521,#70522,#70523,#70524,#70525,#70526,#70527,#70528,#70529,
#70530,#70531,#70532,#70533,#70534,#70535,#70536,#70537,#70538,#70539,#70540,
#70541,#70542,#70543,#70544,#70545,#70546,#70547,#70548,#70549,#70550,#70551,
#70552,#70553,#70554,#70555,#70556,#70557,#70558,#70559,#70560,#70561,#70562,
#70563,#70564,#70565,#70566,#70567,#70568,#70569,#70570,#70571,#70572,#70573,
#70574,#70575,#70576),.UNSPECIFIED.,.F.,.F.,(4,2,2,2,2,2,2,2,2,2,2,2,2,
2,2,2,2,2,2,2,2,2,2,2,2,2,2,2,2,2,2,2,2,2,2,2,2,2,2,2,2,2,2,2,2,2,2,2,2,
2,2,2,2,2,2,2,2,2,2,2,2,2,2,2,2,2,2,2,2,2,2,2,2,2,2,2,2,2,2,2,2,2,2,2,2,
2,2,2,2,2,2,2,2,2,2,2,2,2,2,2,2,2,2,2,2,2,2,2,2,2,2,2,2,4),(-2.66748066396766,
-2.64325165294474,-2.63611998857546,-2.63432914679269,-2.6331142274289,
-2.63210518692895,-2.63103064790152,-2.62964466350476,-2.62674376603921,
-2.59982441801465,-2.58614200050883,-2.57462196577174,-2.54604820313479,
-2.53214899282668,-2.52854547413825,-2.52639366245585,-2.52447447035581,
-2.52204958324415,-2.51731825731717,-2.47994237194092,-2.42958389839601,
-2.42522387950895,-2.42204644301473,-2.42060887408388,-2.4195236539985,
-2.4183371979469,-2.41638144970986,-2.41006037803734,-2.4080000595306,-2.35602879302201,
-2.32315616991477,-2.31773705582591,-2.31520955914026,-2.3132777088833,
-2.31143746612195,-2.30831990111571,-2.29985602604933,-2.29781059032818,
-2.23583608353085,-2.21970622265552,-2.21131263343446,-2.20923883645165,
-2.20802607386156,-2.20694821608152,-2.20555744504906,-2.20324687255974,
-2.18912145936736,-2.18398898501836,-2.14011387655121,-2.10956182064669,
-2.10512208970602,-2.10278932770777,-2.10087736000318,-2.09866094449101,
-2.094865914625,-2.08018098825123,-2.07341156456318,-2.02549659616954,-2.0081840522412,
-1.99938767863716,-1.99728211867183,-1.9960623108214,-1.99498591849885,
-1.99360696590135,-1.99133649089239,-1.97803188926882,-1.9742970159181,
-1.92390847972603,-1.90628290727486,-1.89549845985183,-1.89219648694784,
-1.89011143904926,-1.88817519919052,-1.88566179821301,-1.88146225363339,
-1.85137878627351,-1.79974424985816,-1.78774269885316,-1.78543170571901,
-1.78416692499859,-1.78309618670941,-1.7817589750698,-1.77967491397366,
-1.76959036346571,-1.76409043029117,-1.7566627632639,-1.74315564492008,
-1.71027397103749,-1.69372031343915,-1.68341376853591,-1.68016540386274,
-1.67809204497705,-1.67615115145131,-1.67360943925168,-1.66931294658394,
-1.63409593080558,-1.58485106489426,-1.57547341884819,-1.57332463114969,
-1.57209522158556,-1.5710204609527,-1.56963373723613,-1.56738702422891,
-1.55455413319405,-1.55238811132641,-1.50510774622675,-1.47658362094603,
-1.47017166108594,-1.46746647789825,-1.46550527825293,-1.46371170374019,
-1.46084215261057,-1.45393070740558,-1.40834652030694),.UNSPECIFIED.);
#756=B_SPLINE_CURVE_WITH_KNOTS('',3,(#70578,#70579,#70580,#70581,#70582,
#70583,#70584,#70585,#70586,#70587,#70588,#70589,#70590,#70591,#70592,#70593,
#70594,#70595,#70596,#70597,#70598,#70599,#70600,#70601,#70602,#70603,#70604,
#70605,#70606,#70607,#70608,#70609,#70610,#70611,#70612,#70613,#70614,#70615,
#70616,#70617,#70618,#70619,#70620,#70621,#70622,#70623,#70624,#70625,#70626,
#70627,#70628,#70629,#70630,#70631,#70632,#70633,#70634,#70635,#70636,#70637,
#70638,#70639,#70640,#70641,#70642,#70643,#70644,#70645,#70646,#70647,#70648,
#70649,#70650,#70651,#70652,#70653,#70654,#70655,#70656,#70657,#70658,#70659,
#70660,#70661,#70662,#70663,#70664,#70665,#70666,#70667,#70668,#70669,#70670,
#70671,#70672,#70673,#70674,#70675,#70676,#70677,#70678,#70679,#70680,#70681,
#70682,#70683,#70684,#70685,#70686,#70687,#70688,#70689,#70690,#70691,#70692,
#70693,#70694,#70695,#70696,#70697,#70698,#70699,#70700,#70701,#70702,#70703,
#70704,#70705,#70706,#70707,#70708,#70709,#70710,#70711,#70712,#70713,#70714,
#70715,#70716,#70717,#70718,#70719,#70720,#70721,#70722,#70723,#70724,#70725,
#70726,#70727,#70728,#70729,#70730,#70731,#70732,#70733,#70734,#70735,#70736,
#70737,#70738,#70739,#70740,#70741,#70742,#70743,#70744,#70745,#70746,#70747,
#70748,#70749,#70750,#70751,#70752,#70753,#70754,#70755,#70756,#70757,#70758,
#70759,#70760,#70761,#70762,#70763,#70764,#70765,#70766,#70767,#70768,#70769,
#70770,#70771,#70772,#70773,#70774,#70775,#70776,#70777,#70778,#70779,#70780,
#70781,#70782,#70783,#70784,#70785,#70786,#70787,#70788,#70789,#70790,#70791,
#70792,#70793,#70794,#70795,#70796,#70797,#70798,#70799),.UNSPECIFIED.,
 .F.,.F.,(4,2,2,2,2,2,2,2,2,2,2,2,2,2,2,2,2,2,2,2,2,2,2,2,2,2,2,2,2,2,2,
2,2,2,2,2,2,2,2,2,2,2,2,2,2,2,2,2,2,2,2,2,2,2,2,2,2,2,2,2,2,2,2,2,2,2,2,
2,2,2,2,2,2,2,2,2,2,2,2,2,2,2,2,2,2,2,2,2,2,2,2,2,2,2,2,2,2,2,2,2,2,2,2,
2,2,2,2,2,2,2,4),(-1.2597871053314,-1.25887347369017,-1.25747165391834,
-1.25639225300539,-1.25518557366362,-1.25313941938559,-1.24508186513212,
-1.22990236286778,-1.19000532650871,-1.15896082754083,-1.15473920053375,
-1.15221921376362,-1.15028176133158,-1.14819920279464,-1.14490923784977,
-1.13423538145055,-1.11686367757923,-1.06815910703513,-1.06164421519791,
-1.04902104344771,-1.0467852565193,-1.0454018029575,-1.04432735582621,-1.04309581997592,
-1.04093743820442,-1.03142541094137,-0.982270896994583,-0.94707459333318,
-0.942778177758734,-0.940236518512811,-0.938295658716597,-0.936222328456378,
-0.93297399196045,-0.922667311552972,-0.906115527507918,-0.873263638508922,
-0.860347034121186,-0.83764215987386,-0.834788517686226,-0.833411718799653,
-0.832338022503596,-0.831102361020054,-0.828924860828711,-0.819134785946288,
-0.7702237455661,-0.735106029926622,-0.730811050487319,-0.728269945308957,
-0.726329338426539,-0.724256113342667,-0.721007597131434,-0.710697442888723,
-0.694137318817379,-0.661280543360498,-0.647507728098617,-0.640736120221123,
-0.638932715519826,-0.625194664212764,-0.622903217053436,-0.621518164924736,
-0.620441147562204,-0.619225301156506,-0.617137147897312,-0.608561829424292,
-0.591900724848428,-0.549983861062186,-0.522882171738444,-0.518758559277137,
-0.516267555254865,-0.514334899235427,-0.512240088120757,-0.508893246797823,
-0.497691736551139,-0.479107693233423,-0.436053004741267,-0.413736718190669,
-0.410895310730124,-0.409521024357598,-0.408447687297467,-0.407210628650563,
-0.405026318471844,-0.395132864872299,-0.346315929464636,-0.311232105982675,
-0.306938077712082,-0.304397417376839,-0.302457082306048,-0.300384081761896,
-0.297135779882849,-0.286825146569242,-0.270263150252942,-0.237926861129942,
-0.201815817541599,-0.198960598642569,-0.197583673275514,-0.196557139456272,
-0.195363769522401,-0.193380885957696,-0.190941232363002,-0.18598313874413,
-0.172433471217775,-0.149619114975562,-0.103071362503241,-0.0958751270226328,
-0.092958673276615,-0.0911568740503026,-0.0892033454969263,-0.0865388014388443,
-0.0803612544710696,-0.0537575033662972,-0.000629602941351068),
 .UNSPECIFIED.);
#757=B_SPLINE_CURVE_WITH_KNOTS('',3,(#70800,#70801,#70802,#70803,#70804,
#70805,#70806,#70807,#70808,#70809,#70810,#70811,#70812,#70813,#70814,#70815,
#70816,#70817,#70818,#70819,#70820,#70821,#70822,#70823),.UNSPECIFIED.,
 .F.,.F.,(4,2,2,2,2,2,2,2,2,2,2,4),(-2.667759750698,-2.65970368163532,-2.65534688392438,
-2.65393402192932,-2.65286686819766,-2.65183675354335,-2.65065694971661,
-2.64873191207764,-2.64266693400501,-2.64138504326144,-2.63358536386622,
-2.59350983441696),.UNSPECIFIED.);
#758=B_SPLINE_CURVE_WITH_KNOTS('',3,(#70829,#70830,#70831,#70832,#70833,
#70834,#70835,#70836,#70837,#70838,#70839,#70840,#70841),.UNSPECIFIED.,
 .F.,.F.,(4,3,3,3,4),(114.057240399931,114.163813791282,114.27025049183,
114.376547404602,114.406671945289),.UNSPECIFIED.);
#759=B_SPLINE_CURVE_WITH_KNOTS('',3,(#70842,#70843,#70844,#70845,#70846,
#70847,#70848,#70849,#70850,#70851),.UNSPECIFIED.,.F.,.F.,(4,1,1,1,1,1,
1,4),(114.406674973252,114.866191745616,115.865028195577,116.863864645539,
117.862701095501,118.861537545463,119.860373995425,120.339865638913),
 .UNSPECIFIED.);
#760=B_SPLINE_CURVE_WITH_KNOTS('',3,(#70852,#70853,#70854,#70855,#70856,
#70857,#70858,#70859,#70860,#70861,#70862,#70863,#70864,#70865,#70866,#70867,
#70868,#70869,#70870,#70871,#70872,#70873,#70874,#70875,#70876,#70877,#70878,
#70879,#70880,#70881,#70882,#70883,#70884,#70885,#70886,#70887,#70888,#70889,
#70890,#70891,#70892,#70893,#70894,#70895,#70896,#70897,#70898,#70899,#70900,
#70901,#70902,#70903,#70904,#70905,#70906,#70907,#70908,#70909,#70910,#70911,
#70912,#70913,#70914,#70915,#70916,#70917,#70918,#70919,#70920,#70921,#70922,
#70923,#70924,#70925,#70926,#70927,#70928,#70929,#70930,#70931,#70932,#70933,
#70934,#70935,#70936,#70937,#70938,#70939,#70940,#70941,#70942,#70943,#70944,
#70945,#70946,#70947,#70948,#70949,#70950,#70951,#70952,#70953,#70954,#70955,
#70956,#70957,#70958,#70959,#70960,#70961,#70962,#70963,#70964,#70965,#70966,
#70967,#70968,#70969,#70970,#70971,#70972,#70973,#70974,#70975,#70976,#70977,
#70978,#70979,#70980,#70981,#70982,#70983,#70984,#70985,#70986,#70987,#70988,
#70989,#70990,#70991,#70992,#70993,#70994,#70995,#70996,#70997,#70998,#70999,
#71000,#71001,#71002,#71003,#71004,#71005,#71006,#71007,#71008,#71009,#71010,
#71011,#71012,#71013,#71014,#71015,#71016,#71017,#71018,#71019,#71020,#71021,
#71022,#71023,#71024,#71025,#71026,#71027,#71028,#71029,#71030,#71031,#71032,
#71033,#71034,#71035,#71036,#71037,#71038,#71039,#71040,#71041,#71042,#71043,
#71044,#71045,#71046,#71047,#71048,#71049,#71050,#71051,#71052,#71053,#71054,
#71055,#71056,#71057,#71058,#71059,#71060,#71061,#71062,#71063,#71064,#71065,
#71066,#71067,#71068,#71069,#71070,#71071,#71072,#71073,#71074,#71075,#71076,
#71077,#71078,#71079,#71080,#71081,#71082,#71083,#71084,#71085,#71086,#71087,
#71088,#71089,#71090,#71091,#71092,#71093,#71094,#71095,#71096,#71097,#71098,
#71099,#71100,#71101,#71102,#71103,#71104,#71105,#71106,#71107,#71108,#71109,
#71110,#71111,#71112,#71113,#71114,#71115),.UNSPECIFIED.,.F.,.F.,(4,2,2,
2,2,2,2,2,2,2,2,2,2,2,2,2,2,2,2,2,2,2,2,2,2,2,2,2,2,2,2,2,2,2,2,2,2,2,2,
2,2,2,2,2,2,2,2,2,2,2,2,2,2,2,2,2,2,2,2,2,2,2,2,2,2,2,2,2,2,2,2,2,2,2,2,
2,2,2,2,2,2,2,2,2,2,2,2,2,2,2,2,2,2,2,2,2,2,2,2,2,2,2,2,2,2,2,2,2,2,2,2,
2,2,2,2,2,2,2,2,2,2,2,2,2,2,2,2,2,2,2,2,4),(-2.59350983441696,-2.58039355821006,
-2.56264877629364,-2.55181134345083,-2.54850310221189,-2.54641638655259,
-2.54448017492711,-2.54196904314671,-2.53777818827189,-2.508277658003,-2.46717253757524,
-2.45174120878521,-2.44632784540861,-2.44372939350055,-2.44162299355241,
-2.44041042587091,-2.44040731116854,-2.44040417763524,-2.44040102491068,
-2.440397852994,-2.44039466191649,-2.44039145130121,-2.44038822114729,-2.44038497129897,
-2.44038170150704,-2.44037841173811,-2.44037510156982,-2.44037177123605,
-2.44036843317822,-2.44036508059764,-2.44036170686419,-2.44035830040255,
-2.4393314385167,-2.43795394913262,-2.43509669186788,-2.39901740817715,
-2.36628980770353,-2.34379016539112,-2.33814477880076,-2.33557502850762,
-2.33363682488902,-2.3318096928843,-2.3292661005672,-2.3226142583808,-2.26691048442739,
-2.24278034575134,-2.23193867646507,-2.22969358600825,-2.22844309908252,
-2.22737115902849,-2.22601542419282,-2.22387090179953,-2.21285121490067,
-2.16159321935567,-2.13290046513907,-2.12646864493506,-2.12376024625422,
-2.12179859010036,-2.12000588793617,-2.11714053969733,-2.11025374837044,
-2.0572080144364,-2.03127863070266,-2.01996567469318,-2.01769283270307,
-2.01643632406596,-2.01536497154924,-2.01401730709105,-2.01139607875927,
-1.99536032524404,-1.99002589608921,-1.97547612193418,-1.94258372428966,
-1.92601689493743,-1.9157044252239,-1.91245540419634,-1.91038191733261,
-1.908441108381,-1.90589980181412,-1.90160465573686,-1.86648816611598,-1.81757147313822,
-1.80781339684992,-1.80563798745994,-1.80440272547343,-1.80332887745643,
-1.80195122229711,-1.79909354371259,-1.7631415572081,-1.73036511925745,
-1.7077923314465,-1.70213677580606,-1.69956499870042,-1.69762632517493,
-1.69579952824608,-1.69325765124335,-1.6866177528121,-1.63078270198163,
-1.59793943797146,-1.59439319603278,-1.59288897697062,-1.59179757900628,
-1.59077020803701,-1.58901999167604,-1.58424099456079,-1.54706883524457,
-1.49680343343329,-1.4904016602027,-1.48769817383609,-1.48573725673049,
-1.48394328737112,-1.4810716798851,-1.47414791125047,-1.42158311608298,
-1.39531119760009,-1.38391089336196,-1.38163289024548,-1.38037518312162,
-1.37930381140584,-1.37795739799209,-1.37534234651273,-1.35942301201897,
-1.35492117671423,-1.33435975724735,-1.2860094575818,-1.27886102805064,
-1.275952021756,-1.27415116971881,-1.2721957871066,-1.26952353577656,-1.2633045979713,
-1.25983685653957),.UNSPECIFIED.);
#761=B_SPLINE_CURVE_WITH_KNOTS('',3,(#71121,#71122,#71123,#71124,#71125,
#71126,#71127,#71128,#71129,#71130,#71131,#71132,#71133,#71134,#71135,#71136,
#71137,#71138,#71139,#71140),.UNSPECIFIED.,.F.,.F.,(4,2,2,2,2,2,2,2,2,4),
(-0.0747504723290347,-0.06102294006139,-0.0562870052721474,-0.0545435820400614,
-0.0535177062400768,-0.052425793662566,-0.0509174408111615,-0.0492296223280002,
-0.0462824121917821,-0.00062912049210774),.UNSPECIFIED.);
#762=B_SPLINE_CURVE_WITH_KNOTS('',3,(#71141,#71142,#71143,#71144,#71145,
#71146,#71147,#71148,#71149,#71150,#71151,#71152,#71153,#71154,#71155,#71156,
#71157,#71158,#71159,#71160,#71161,#71162,#71163,#71164,#71165,#71166,#71167,
#71168,#71169,#71170,#71171,#71172,#71173,#71174,#71175,#71176,#71177,#71178,
#71179,#71180,#71181,#71182,#71183,#71184,#71185,#71186,#71187,#71188,#71189,
#71190,#71191,#71192,#71193,#71194,#71195,#71196,#71197,#71198,#71199,#71200,
#71201,#71202,#71203,#71204,#71205,#71206,#71207,#71208,#71209,#71210,#71211,
#71212,#71213,#71214,#71215,#71216,#71217,#71218,#71219,#71220,#71221,#71222,
#71223,#71224,#71225,#71226,#71227,#71228,#71229,#71230,#71231,#71232,#71233,
#71234,#71235,#71236,#71237,#71238,#71239,#71240,#71241,#71242,#71243,#71244,
#71245,#71246,#71247,#71248,#71249,#71250,#71251,#71252,#71253,#71254,#71255,
#71256,#71257,#71258,#71259,#71260,#71261,#71262,#71263,#71264,#71265,#71266,
#71267,#71268,#71269,#71270,#71271,#71272,#71273,#71274,#71275,#71276,#71277,
#71278,#71279,#71280,#71281,#71282,#71283,#71284,#71285,#71286,#71287,#71288,
#71289,#71290,#71291,#71292,#71293,#71294,#71295,#71296,#71297,#71298,#71299,
#71300,#71301,#71302,#71303,#71304,#71305,#71306,#71307,#71308,#71309,#71310,
#71311,#71312,#71313,#71314,#71315,#71316,#71317,#71318,#71319,#71320,#71321),
 .UNSPECIFIED.,.F.,.F.,(4,3,3,3,3,3,3,3,3,3,3,3,3,3,3,3,3,3,3,3,3,3,3,3,
3,3,3,3,3,3,3,3,3,3,3,3,3,3,3,3,3,3,3,3,3,3,3,3,3,3,3,3,3,3,3,3,3,3,3,3,
4),(108.12348663811,108.225421296431,108.327291076164,108.429131491865,
108.530978014042,108.632930880402,108.734945943836,108.837130903885,108.873173045844,
108.976567782892,109.079809065007,109.182929030399,109.285983598608,109.389006806966,
109.492032649639,109.595165416417,109.698354507827,109.801726501209,109.872009495806,
109.975404232854,110.078645514969,110.181765480362,110.284820048571,110.387843256929,
110.490869099601,110.594001866379,110.69719095779,110.800562951171,110.870845945768,
110.974240682816,111.077481964931,111.180601930323,111.283656498532,111.38667970689,
111.489705549562,111.592838316341,111.69602740775,111.799399401132,111.86968239573,
111.973077132778,112.076318414893,112.179438380285,112.282492948494,112.385516156852,
112.488541999524,112.591674766302,112.694863857712,112.798235851094,112.868518845692,
112.97191358274,113.075154864856,113.178274830248,113.281329398457,113.384352606815,
113.487378449487,113.590511216266,113.693700307675,113.797072301057,113.867355295654,
113.974272639397,114.057240399931),.UNSPECIFIED.);
#763=B_SPLINE_CURVE_WITH_KNOTS('',3,(#71323,#71324,#71325,#71326,#71327,
#71328,#71329,#71330,#71331,#71332,#71333,#71334,#71335,#71336,#71337,#71338,
#71339,#71340,#71341,#71342,#71343,#71344,#71345,#71346,#71347,#71348,#71349,
#71350,#71351,#71352,#71353,#71354,#71355,#71356,#71357,#71358,#71359,#71360,
#71361,#71362,#71363,#71364,#71365,#71366,#71367,#71368,#71369,#71370,#71371,
#71372,#71373,#71374,#71375,#71376,#71377,#71378,#71379,#71380,#71381,#71382,
#71383,#71384,#71385,#71386,#71387,#71388,#71389,#71390,#71391,#71392,#71393,
#71394,#71395,#71396,#71397,#71398,#71399,#71400,#71401,#71402,#71403,#71404,
#71405,#71406,#71407,#71408,#71409,#71410,#71411,#71412,#71413,#71414,#71415,
#71416,#71417,#71418,#71419,#71420,#71421,#71422,#71423,#71424,#71425,#71426,
#71427,#71428,#71429,#71430,#71431,#71432,#71433,#71434,#71435,#71436,#71437,
#71438,#71439,#71440,#71441,#71442,#71443,#71444,#71445,#71446,#71447,#71448,
#71449,#71450,#71451,#71452,#71453,#71454,#71455,#71456,#71457,#71458,#71459,
#71460,#71461,#71462,#71463,#71464,#71465,#71466,#71467,#71468,#71469,#71470,
#71471,#71472,#71473,#71474,#71475,#71476,#71477,#71478,#71479,#71480,#71481,
#71482,#71483,#71484,#71485,#71486,#71487,#71488,#71489,#71490,#71491,#71492,
#71493,#71494,#71495,#71496,#71497,#71498,#71499,#71500,#71501,#71502,#71503,
#71504,#71505,#71506,#71507,#71508,#71509,#71510,#71511,#71512,#71513,#71514,
#71515,#71516,#71517,#71518,#71519,#71520,#71521,#71522,#71523,#71524,#71525,
#71526,#71527,#71528,#71529,#71530,#71531,#71532,#71533,#71534,#71535,#71536,
#71537,#71538),.UNSPECIFIED.,.F.,.F.,(4,2,2,2,2,2,2,2,2,2,2,2,2,2,2,2,2,
2,2,2,2,2,2,2,2,2,2,2,2,2,2,2,2,2,2,2,2,2,2,2,2,2,2,2,2,2,2,2,2,2,2,2,2,
2,2,2,2,2,2,2,2,2,2,2,2,2,2,2,2,2,2,2,2,2,2,2,2,2,2,2,2,2,2,2,2,2,2,2,2,
2,2,2,2,2,2,2,2,2,2,2,2,2,2,2,2,2,2,4),(-1.25983685653957,-1.2363744642156,
-1.1958522808464,-1.17286244743288,-1.17000730397881,-1.1686301350547,-1.16755631675952,
-1.16632070299258,-1.16414373713736,-1.15436352877039,-1.10543890910008,
-1.07031498195434,-1.06601956755178,-1.06347821694089,-1.06153742948484,
-1.05946401813863,-1.05621522396254,-1.04590430459282,-1.02934306292726,
-0.996483599797937,-0.982742350350651,-0.975892406261312,-0.975578869095316,
-0.970007428554194,-0.959995609972315,-0.95791662584862,-0.95658099402074,
-0.955510371164392,-0.954244384698694,-0.951927683705647,-0.93981815029731,
-0.887088451149664,-0.876442966387558,-0.857376854613134,-0.853613472599162,
-0.851204245472093,-0.849286724526475,-0.84712543589334,-0.84347871972519,
-0.82905929736825,-0.778655873958179,-0.748982408997737,-0.746068394828556,
-0.744679858434579,-0.743605047970853,-0.74237710627218,-0.740234444215214,
-0.730939049319063,-0.712090773430482,-0.671644321247857,-0.659367695302661,
-0.644790071409047,-0.641004701799636,-0.638790609095994,-0.636878637071265,
-0.634543345405316,-0.630091033724474,-0.599061232992771,-0.55110113604688,
-0.536504623440271,-0.534172221810807,-0.532775089796961,-0.531696456253336,
-0.530487467068014,-0.528430413770078,-0.520240202580606,-0.504687456620258,
-0.463145707466814,-0.434210277073354,-0.430031719140513,-0.427524515873234,
-0.425589300708636,-0.423501647145032,-0.420187609892399,-0.409292201123117,
-0.391415722944751,-0.340792529831821,-0.324645112217682,-0.322019930743042,
-0.320671450254275,-0.319600087051743,-0.318344310563733,-0.316074671633414,
-0.304816503315135,-0.27909797100561,-0.225709947894199,-0.218851080843394,
-0.216045375303452,-0.21408523103112,-0.212146031668788,-0.210185549506391,
-0.205109051866494,-0.163990473157819,-0.115019701111411,-0.110791357719309,
-0.109127238460932,-0.108116689967441,-0.107013221161621,-0.105442050010592,
-0.10148989773849,-0.0819023791992277,-0.0267279003317656,-0.0187639987473031,
-0.00802108770802645,-0.00466632887790808,-0.0025813007720164,-0.00128118372687951,
-0.000628942024347663),.UNSPECIFIED.);
#764=B_SPLINE_CURVE_WITH_KNOTS('',3,(#71539,#71540,#71541,#71542,#71543,
#71544,#71545,#71546,#71547,#71548,#71549,#71550,#71551),.UNSPECIFIED.,
 .F.,.F.,(4,3,3,3,4),(-104.372003947921,-104.263735348717,-104.155311094171,
-104.046631225627,-104.022525439493),.UNSPECIFIED.);
#765=B_SPLINE_CURVE_WITH_KNOTS('',3,(#71556,#71557,#71558,#71559,#71560,
#71561,#71562,#71563,#71564,#71565,#71566,#71567,#71568,#71569,#71570,#71571,
#71572,#71573,#71574,#71575,#71576,#71577,#71578,#71579,#71580,#71581,#71582,
#71583,#71584,#71585,#71586,#71587,#71588,#71589,#71590,#71591,#71592,#71593,
#71594,#71595,#71596,#71597,#71598,#71599,#71600,#71601,#71602,#71603,#71604,
#71605,#71606,#71607,#71608,#71609,#71610,#71611,#71612,#71613,#71614,#71615,
#71616,#71617,#71618,#71619,#71620,#71621,#71622,#71623,#71624,#71625,#71626,
#71627,#71628,#71629,#71630,#71631,#71632,#71633,#71634,#71635,#71636,#71637,
#71638,#71639,#71640,#71641,#71642,#71643,#71644,#71645,#71646,#71647,#71648,
#71649,#71650,#71651,#71652,#71653,#71654,#71655,#71656,#71657,#71658,#71659,
#71660,#71661,#71662,#71663,#71664,#71665,#71666,#71667,#71668,#71669,#71670,
#71671,#71672,#71673,#71674,#71675,#71676,#71677,#71678,#71679,#71680,#71681,
#71682,#71683,#71684,#71685,#71686,#71687,#71688,#71689,#71690,#71691,#71692,
#71693,#71694,#71695,#71696,#71697,#71698,#71699,#71700,#71701,#71702,#71703,
#71704,#71705,#71706,#71707,#71708,#71709,#71710,#71711,#71712,#71713,#71714,
#71715,#71716,#71717,#71718,#71719,#71720,#71721,#71722,#71723,#71724,#71725,
#71726,#71727,#71728,#71729,#71730,#71731,#71732,#71733,#71734,#71735,#71736,
#71737,#71738,#71739,#71740,#71741,#71742,#71743,#71744,#71745,#71746,#71747,
#71748,#71749,#71750,#71751,#71752,#71753,#71754,#71755,#71756,#71757,#71758,
#71759,#71760,#71761,#71762,#71763,#71764,#71765,#71766,#71767,#71768,#71769,
#71770,#71771,#71772,#71773,#71774,#71775),.UNSPECIFIED.,.F.,.F.,(4,2,2,
2,2,2,2,2,2,2,2,2,2,2,2,2,2,2,2,2,2,2,2,2,2,2,2,2,2,2,2,2,2,2,2,2,2,2,2,
2,2,2,2,2,2,2,2,2,2,2,2,2,2,2,2,2,2,2,2,2,2,2,2,2,2,2,2,2,2,2,2,2,2,2,2,
2,2,2,2,2,2,2,2,2,2,2,2,2,2,2,2,2,2,2,2,2,2,2,2,2,2,2,2,2,2,2,2,2,2,4),
(-1.40835488213934,-1.37307257504326,-1.3339620916423,-1.33297753375494,
-1.32826981672132,-1.32653033786744,-1.32550501098063,-1.32441218079595,
-1.3229001105707,-1.31930847814899,-1.28016936056107,-1.23134352087163,
-1.22421237079347,-1.22130613403507,-1.21950569928475,-1.21754974510166,
-1.21487486720901,-1.20864139691479,-1.18159511324464,-1.14086737517617,
-1.11820862392735,-1.11535573440555,-1.11397894781042,-1.11290509602158,
-1.11166906909407,-1.10949047827219,-1.09968808257067,-1.05077792159248,
-1.01565733517771,-1.01136168157912,-1.00882016567859,-1.00687923830419,
-1.00480566420508,-1.0015565873001,-0.991244536980126,-0.97468125662034,
-0.941818686606974,-0.928011069381496,-0.921314234906394,-0.905865126248385,
-0.903497163203982,-0.902089567451067,-0.90100940943892,-0.899805967893813,
-0.897774199595886,-0.889884364618558,-0.875168237518788,-0.846104164476846,
-0.803698149152738,-0.799404687404572,-0.796863863883766,-0.794923117079057,
-0.792849398195703,-0.78959938910586,-0.77927842973857,-0.762695175853825,
-0.72981688302325,-0.714515615030122,-0.709793792620108,-0.693941565195866,
-0.691328752708666,-0.689982895750886,-0.688911651900714,-0.687653734986515,
-0.685374423961639,-0.673948890377299,-0.647572514827088,-0.595122290095803,
-0.588188793898627,-0.585315750368055,-0.583521643686318,-0.581561191357775,
-0.578859462281914,-0.572467091064481,-0.526046239066656,-0.484947967846882,
-0.480263104017284,-0.478527321164545,-0.477502870249328,-0.476409866291896,
-0.47489574639119,-0.471290890966269,-0.432950716683481,-0.38331732109614,
-0.376221647411313,-0.373321726606491,-0.371522734313794,-0.369566391628544,
-0.366887452921059,-0.360806545645847,-0.352445678521271,-0.301551117062902,
-0.270313242225972,-0.26740127492247,-0.266013098083552,-0.264938282463211,
-0.263710017758472,-0.261566049314298,-0.252414971273518,-0.20366644528238,
-0.167704290585459,-0.162982356767182,-0.160559558506669,-0.158640677246885,
-0.15648780368554,-0.154258048649232,-0.146612097675678,-0.121083045893507,
-0.100337618335071,-0.0747504723290347),.UNSPECIFIED.);
#766=B_SPLINE_CURVE_WITH_KNOTS('',3,(#71777,#71778,#71779,#71780,#71781,
#71782,#71783,#71784,#71785,#71786,#71787,#71788,#71789,#71790,#71791,#71792,
#71793,#71794,#71795,#71796,#71797,#71798,#71799,#71800,#71801,#71802,#71803,
#71804,#71805,#71806,#71807,#71808,#71809,#71810,#71811,#71812,#71813,#71814,
#71815,#71816,#71817,#71818,#71819,#71820,#71821,#71822,#71823,#71824,#71825,
#71826,#71827,#71828,#71829,#71830,#71831,#71832,#71833,#71834,#71835,#71836,
#71837,#71838,#71839,#71840,#71841,#71842,#71843,#71844,#71845,#71846,#71847,
#71848,#71849,#71850,#71851,#71852,#71853,#71854,#71855,#71856,#71857,#71858,
#71859,#71860,#71861,#71862,#71863,#71864,#71865,#71866,#71867,#71868,#71869,
#71870,#71871,#71872,#71873,#71874,#71875,#71876,#71877,#71878,#71879,#71880,
#71881,#71882,#71883,#71884,#71885,#71886,#71887,#71888,#71889,#71890,#71891,
#71892,#71893,#71894,#71895,#71896,#71897,#71898,#71899,#71900,#71901,#71902,
#71903,#71904,#71905,#71906,#71907,#71908,#71909,#71910,#71911,#71912,#71913,
#71914,#71915,#71916,#71917,#71918,#71919,#71920,#71921,#71922,#71923,#71924,
#71925,#71926,#71927,#71928,#71929,#71930,#71931,#71932,#71933,#71934,#71935,
#71936,#71937,#71938,#71939,#71940,#71941,#71942,#71943,#71944,#71945,#71946,
#71947,#71948,#71949,#71950,#71951,#71952,#71953,#71954,#71955,#71956,#71957),
 .UNSPECIFIED.,.F.,.F.,(4,3,3,3,3,3,3,3,3,3,3,3,3,3,3,3,3,3,3,3,3,3,3,3,
3,3,3,3,3,3,3,3,3,3,3,3,3,3,3,3,3,3,3,3,3,3,3,3,3,3,3,3,3,3,3,3,3,3,3,3,
4),(-104.022525439493,-103.9135142963,-103.878990796035,-103.775596058987,
-103.672354776872,-103.569234811479,-103.46618024327,-103.363157034913,
-103.26013119224,-103.156998425462,-103.053809334052,-102.95043734067,-102.880154346073,
-102.776759609025,-102.67351832691,-102.570398361518,-102.467343793309,
-102.364320584951,-102.261294742278,-102.1581619755,-102.054972884091,-101.951600890709,
-101.881317896111,-101.777923159063,-101.674681876948,-101.571561911556,
-101.468507343347,-101.365484134989,-101.262458292316,-101.159325525538,
-101.056136434128,-100.952764440747,-100.882481446149,-100.779086709101,
-100.675845426986,-100.572725461594,-100.469670893385,-100.366647685027,
-100.263621842355,-100.160489075577,-100.057299984167,-99.9539279907856,
-99.8836449961874,-99.7802502591395,-99.6770089770246,-99.5738890116324,
-99.4708344434235,-99.3678112350658,-99.2647853923933,-99.1616526256152,
-99.0584635342055,-98.9550915408238,-98.8848085462256,-98.7829332776308,
-98.6811932844012,-98.579552537636,-98.4779751499172,-98.3763829554482,
-98.2747883682234,-98.1730805291731,-98.0888188327757),.UNSPECIFIED.);
#767=B_SPLINE_CURVE_WITH_KNOTS('',3,(#71958,#71959,#71960,#71961,#71962),
 .UNSPECIFIED.,.F.,.F.,(4,1,4),(-98.0888186411165,-97.8859720962637,-97.7379483049134),
 .UNSPECIFIED.);
#768=B_SPLINE_CURVE_WITH_KNOTS('',3,(#71968,#71969,#71970,#71971,#71972,
#71973,#71974,#71975,#71976,#71977,#71978,#71979,#71980,#71981,#71982,#71983,
#71984,#71985,#71986,#71987,#71988,#71989),.UNSPECIFIED.,.F.,.F.,(4,2,2,
2,2,2,2,2,2,2,4),(-0.0750517038529886,-0.0634020312911012,-0.0604357711843507,
-0.0436144622418274,-0.0399995473077869,-0.0376361122359522,-0.0357225144891595,
-0.0339209951592301,-0.0317709072211862,-0.0286342749703805,-0.000628476579351984),
 .UNSPECIFIED.);
#769=B_SPLINE_CURVE_WITH_KNOTS('',3,(#71990,#71991,#71992,#71993,#71994,
#71995,#71996,#71997,#71998,#71999,#72000,#72001,#72002,#72003,#72004,#72005,
#72006,#72007,#72008,#72009,#72010,#72011,#72012,#72013,#72014,#72015,#72016,
#72017,#72018,#72019,#72020,#72021,#72022,#72023,#72024,#72025,#72026,#72027,
#72028,#72029,#72030,#72031,#72032,#72033,#72034,#72035,#72036,#72037,#72038,
#72039,#72040,#72041,#72042,#72043,#72044,#72045,#72046,#72047,#72048,#72049,
#72050,#72051,#72052,#72053,#72054,#72055,#72056,#72057,#72058,#72059,#72060,
#72061,#72062,#72063,#72064,#72065,#72066,#72067,#72068,#72069,#72070,#72071,
#72072,#72073,#72074,#72075,#72076,#72077,#72078,#72079,#72080,#72081,#72082,
#72083,#72084,#72085,#72086,#72087,#72088,#72089,#72090,#72091,#72092,#72093,
#72094,#72095,#72096,#72097,#72098,#72099,#72100,#72101,#72102,#72103,#72104,
#72105,#72106,#72107,#72108,#72109,#72110,#72111,#72112,#72113,#72114,#72115,
#72116,#72117,#72118,#72119,#72120,#72121,#72122,#72123,#72124,#72125,#72126,
#72127,#72128,#72129,#72130,#72131,#72132,#72133,#72134,#72135,#72136,#72137,
#72138,#72139,#72140,#72141,#72142,#72143,#72144,#72145,#72146,#72147,#72148,
#72149,#72150,#72151,#72152,#72153,#72154,#72155,#72156,#72157,#72158,#72159,
#72160,#72161,#72162,#72163,#72164,#72165,#72166,#72167,#72168,#72169,#72170,
#72171,#72172,#72173,#72174,#72175,#72176,#72177,#72178,#72179,#72180,#72181,
#72182,#72183,#72184,#72185,#72186,#72187,#72188,#72189,#72190,#72191,#72192,
#72193,#72194,#72195,#72196,#72197,#72198,#72199,#72200,#72201,#72202,#72203,
#72204,#72205,#72206,#72207,#72208,#72209,#72210,#72211,#72212,#72213),
 .UNSPECIFIED.,.F.,.F.,(4,2,2,2,2,2,2,2,2,2,2,2,2,2,2,2,2,2,2,2,2,2,2,2,
2,2,2,2,2,2,2,2,2,2,2,2,2,2,2,2,2,2,2,2,2,2,2,2,2,2,2,2,2,2,2,2,2,2,2,2,
2,2,2,2,2,2,2,2,2,2,2,2,2,2,2,2,2,2,2,2,2,2,2,2,2,2,2,2,2,2,2,2,2,2,2,2,
2,2,2,2,2,2,2,2,2,2,2,2,2,2,2,4),(-2.66756143460973,-2.63526158114188,-2.61196230848377,
-2.60134680143366,-2.59911541518788,-2.59786784425495,-2.59679548087336,
-2.59543544972892,-2.59275695546045,-2.57521180506395,-2.56873788357839,
-2.52873913767827,-2.50908323364963,-2.50137439649208,-2.49567141392468,
-2.4930937964052,-2.49114560662755,-2.48933460017414,-2.48637121157221,
-2.47890392946452,-2.43049268194267,-2.39142719262711,-2.38785262315977,
-2.38634352320541,-2.38525126065573,-2.38422520908087,-2.38248181364631,
-2.37774784605682,-2.33778536583976,-2.29024389770352,-2.28384709393534,
-2.28114439637311,-2.27918357379278,-2.27738936151038,-2.27451664630728,
-2.26758649178128,-2.21511242539049,-2.18877416132953,-2.17735697994162,
-2.17507796411341,-2.17382001241067,-2.17274862275564,-2.17140242886039,
-2.16878851328827,-2.15290786883536,-2.14823494534728,-2.1076598964018,
-2.07837184499827,-2.07186899357031,-2.0691483656054,-2.0671842174186,-2.06539359761044,
-2.06254101658788,-2.05573352895158,-2.00168838114947,-1.97643617187404,
-1.96529679649396,-1.96303373522922,-1.96177921650124,-1.96070747757425,
-1.95935666877263,-1.95672147233761,-1.94033577505885,-1.93130037954646,
-1.89233437778975,-1.86585523809554,-1.85969238780467,-1.85702970978129,
-1.85507586639276,-1.85327259845599,-1.85035112192351,-1.8431294203899,
-1.79878562848196,-1.78472886360406,-1.76327485952442,-1.75318358713273,
-1.75098562471165,-1.74974532232207,-1.74867201891863,-1.74730146858214,
-1.74510858042782,-1.73333797761026,-1.72962678752198,-1.72236562682105,
-1.67901010237693,-1.66042269618648,-1.64921988866115,-1.64587222689119,
-1.64377681315624,-1.64184354124563,-1.63935166085027,-1.63522644810675,
-1.60809059376719,-1.56616640321535,-1.54954738484282,-1.54098479943008,
-1.53889724862778,-1.53768130974134,-1.53660391771465,-1.53521799319194,
-1.53292428769805,-1.51915035535241,-1.50784475531045,-1.46844818339477,
-1.4418753908946,-1.43570088024064,-1.43303617244619,-1.43108197182575,
-1.42927916916287,-1.42636022261411,-1.41915355869009,-1.40835488213934),
 .UNSPECIFIED.);
#770=B_SPLINE_CURVE_WITH_KNOTS('',3,(#72215,#72216,#72217,#72218,#72219,
#72220,#72221,#72222,#72223,#72224),.UNSPECIFIED.,.F.,.F.,(4,1,1,1,1,1,
1,4),(-97.7379483049134,-96.8871356463018,-95.88829919634,-94.8894627463781,
-93.8906262964162,-92.8917898464543,-91.8929533964925,-91.8056333339369),
 .UNSPECIFIED.);
#771=B_SPLINE_CURVE_WITH_KNOTS('',3,(#72225,#72226,#72227,#72228,#72229,
#72230,#72231,#72232),.UNSPECIFIED.,.F.,.F.,(4,2,2,4),(-2.66774030490623,
-2.61554842952445,-2.59714695246637,-2.59330484294858),.UNSPECIFIED.);
#772=B_SPLINE_CURVE_WITH_KNOTS('',3,(#72237,#72238,#72239,#72240,#72241,
#72242,#72243,#72244,#72245,#72246,#72247,#72248,#72249,#72250,#72251,#72252,
#72253,#72254,#72255,#72256,#72257,#72258,#72259,#72260,#72261,#72262,#72263,
#72264,#72265,#72266,#72267,#72268,#72269,#72270,#72271,#72272,#72273,#72274,
#72275,#72276,#72277,#72278,#72279,#72280,#72281,#72282,#72283,#72284,#72285,
#72286,#72287,#72288,#72289,#72290,#72291,#72292,#72293,#72294,#72295,#72296,
#72297,#72298,#72299,#72300,#72301,#72302,#72303,#72304,#72305,#72306,#72307,
#72308,#72309,#72310,#72311,#72312,#72313,#72314,#72315,#72316,#72317,#72318,
#72319,#72320,#72321,#72322,#72323,#72324,#72325,#72326,#72327,#72328,#72329,
#72330,#72331,#72332,#72333,#72334,#72335,#72336,#72337,#72338,#72339,#72340,
#72341,#72342,#72343,#72344,#72345,#72346,#72347,#72348,#72349,#72350,#72351,
#72352,#72353,#72354,#72355,#72356,#72357,#72358,#72359,#72360,#72361,#72362,
#72363,#72364,#72365,#72366,#72367,#72368,#72369,#72370,#72371,#72372,#72373,
#72374,#72375,#72376,#72377,#72378,#72379,#72380,#72381,#72382,#72383,#72384,
#72385,#72386,#72387,#72388,#72389,#72390,#72391,#72392,#72393,#72394,#72395,
#72396,#72397,#72398,#72399,#72400,#72401,#72402,#72403,#72404,#72405,#72406,
#72407,#72408,#72409,#72410,#72411,#72412,#72413,#72414,#72415,#72416,#72417,
#72418,#72419,#72420,#72421,#72422,#72423,#72424,#72425,#72426,#72427,#72428,
#72429,#72430,#72431,#72432,#72433,#72434,#72435,#72436,#72437,#72438,#72439,
#72440,#72441,#72442,#72443,#72444,#72445,#72446,#72447,#72448,#72449,#72450,
#72451,#72452),.UNSPECIFIED.,.F.,.F.,(4,2,2,2,2,2,2,2,2,2,2,2,2,2,2,2,2,
2,2,2,2,2,2,2,2,2,2,2,2,2,2,2,2,2,2,2,2,2,2,2,2,2,2,2,2,2,2,2,2,2,2,2,2,
2,2,2,2,2,2,2,2,2,2,2,2,2,2,2,2,2,2,2,2,2,2,2,2,2,2,2,2,2,2,2,2,2,2,2,2,
2,2,2,2,2,2,2,2,2,2,2,2,2,2,2,2,2,2,4),(-1.40856908540218,-1.37753522697878,
-1.33437646265475,-1.31573881175565,-1.31200609447521,-1.3096061864511,
-1.30768941851849,-1.30552186708829,-1.30184727203203,-1.2870843685882,
-1.25915934386313,-1.20936241991539,-1.20515946999307,-1.20349949633772,
-1.20248970435662,-1.20138546249729,-1.19981047693733,-1.19583457286336,
-1.17602191091469,-1.14710912276,-1.10479019933331,-1.10049508706726,-1.09795384795708,
-1.09601310691878,-1.09393970760558,-1.0906908538647,-1.08037908431328,
-1.06381584829322,-1.03095508345967,-1.01703053161134,-1.01060083943746,
-0.995017829819212,-0.992416282823265,-0.991072895883222,-0.990001854157967,
-0.988742123099013,-0.986454275545898,-0.974875690663942,-0.947884200897821,
-0.896303812276763,-0.889312873156469,-0.886430427292855,-0.88463466695291,
-0.882675776730312,-0.879982340662421,-0.873638322814003,-0.845680030525046,
-0.799188271842068,-0.783069666423301,-0.78044234287599,-0.779093421705149,
-0.778022054296434,-0.776766673285566,-0.77449876366209,-0.763269746460913,
-0.737664174487258,-0.684114700678137,-0.677265839950885,-0.674406855721565,
-0.672615400618229,-0.670652911279771,-0.667939314949484,-0.661475881210283,
-0.607416520889947,-0.571354708571906,-0.568495766685227,-0.567117978027443,
-0.566044245810071,-0.564809373611564,-0.562635250243668,-0.552893181014568,
-0.503945162920013,-0.468810091673628,-0.464518828287601,-0.461978880853651,
-0.460038558400026,-0.457965055434286,-0.454714888497141,-0.444389237321866,
-0.427794453298269,-0.371095860345277,-0.358711505310279,-0.356488685664063,
-0.355109269256772,-0.35403539081567,-0.352801615436594,-0.350632439144015,
-0.340961945140005,-0.291953827328591,-0.256811972815142,-0.252513674847289,
-0.249971703843863,-0.248031067492687,-0.24624041893856,-0.243302997727772,
-0.235328228390283,-0.223523979421678,-0.190998868263142,-0.150078454373832,
-0.145387647649334,-0.143651117531566,-0.142626623837441,-0.141533912861887,
-0.140020751969381,-0.136420736347178,-0.0985299881454376,-0.0757357797478958,
-0.0750517038529886),.UNSPECIFIED.);
#773=B_SPLINE_CURVE_WITH_KNOTS('',3,(#72453,#72454,#72455,#72456,#72457,
#72458,#72459,#72460,#72461,#72462,#72463,#72464,#72465,#72466,#72467,#72468,
#72469,#72470,#72471,#72472,#72473,#72474,#72475,#72476,#72477,#72478,#72479,
#72480,#72481,#72482,#72483,#72484,#72485,#72486,#72487,#72488,#72489,#72490,
#72491,#72492,#72493,#72494,#72495,#72496,#72497,#72498,#72499,#72500,#72501,
#72502,#72503,#72504,#72505,#72506,#72507,#72508,#72509,#72510,#72511,#72512,
#72513,#72514,#72515,#72516,#72517,#72518,#72519,#72520,#72521,#72522,#72523,
#72524,#72525,#72526,#72527,#72528,#72529,#72530,#72531,#72532,#72533,#72534,
#72535,#72536,#72537,#72538,#72539,#72540,#72541,#72542,#72543,#72544,#72545,
#72546,#72547,#72548,#72549,#72550,#72551,#72552,#72553,#72554,#72555,#72556,
#72557,#72558,#72559,#72560,#72561,#72562,#72563,#72564,#72565,#72566,#72567,
#72568,#72569,#72570,#72571,#72572,#72573,#72574,#72575,#72576,#72577,#72578,
#72579,#72580,#72581,#72582,#72583,#72584,#72585,#72586,#72587,#72588,#72589,
#72590,#72591,#72592,#72593,#72594,#72595,#72596,#72597,#72598,#72599,#72600,
#72601,#72602,#72603,#72604,#72605,#72606,#72607,#72608,#72609,#72610,#72611,
#72612,#72613,#72614,#72615,#72616,#72617,#72618,#72619,#72620,#72621,#72622,
#72623,#72624,#72625,#72626,#72627,#72628,#72629,#72630,#72631,#72632,#72633,
#72634,#72635,#72636,#72637,#72638,#72639,#72640,#72641,#72642,#72643,#72644,
#72645,#72646,#72647,#72648,#72649,#72650,#72651,#72652,#72653,#72654,#72655,
#72656,#72657,#72658,#72659,#72660,#72661,#72662,#72663,#72664,#72665,#72666,
#72667,#72668,#72669,#72670,#72671,#72672,#72673,#72674,#72675,#72676,#72677,
#72678,#72679,#72680,#72681,#72682,#72683,#72684,#72685,#72686,#72687,#72688,
#72689,#72690,#72691,#72692,#72693,#72694,#72695,#72696,#72697,#72698,#72699,
#72700,#72701,#72702,#72703,#72704,#72705,#72706,#72707,#72708,#72709,#72710,
#72711,#72712,#72713,#72714,#72715,#72716,#72717,#72718,#72719,#72720,#72721,
#72722,#72723,#72724,#72725,#72726,#72727,#72728,#72729,#72730,#72731,#72732,
#72733,#72734,#72735,#72736,#72737,#72738,#72739,#72740,#72741,#72742),
 .UNSPECIFIED.,.F.,.F.,(4,2,2,2,2,2,2,2,2,2,2,2,2,2,2,2,2,2,2,2,2,2,2,2,
2,2,2,2,2,2,2,2,2,2,2,2,2,2,2,2,2,2,2,2,2,2,2,2,2,2,2,2,2,2,2,2,2,2,2,2,
2,2,2,2,2,2,2,2,2,2,2,2,2,2,2,2,2,2,2,2,2,2,2,2,2,2,2,2,2,2,2,2,2,2,2,2,
2,2,2,2,2,2,2,2,2,2,2,2,2,2,2,2,2,2,2,2,2,2,2,2,2,2,2,2,2,2,2,2,2,2,2,2,
2,2,2,2,2,2,2,2,2,2,2,2,4),(-2.59330484294858,-2.58602528648615,-2.58268708564519,
-2.58059427506186,-2.57866114609222,-2.57616628761683,-2.57202929296363,
-2.54438681825075,-2.50209974648873,-2.48614458575997,-2.48061017196621,
-2.47797051539189,-2.47585511611322,-2.47463186447299,-2.47462831875154,
-2.47462475941621,-2.47462118639474,-2.47461759969858,-2.47461399899299,
-2.47461010811779,-2.47460614934466,-2.47460212124373,-2.47459802244419,
-2.47459385135599,-2.47458960644169,-2.47458528604957,-2.47458088858814,
-2.47457641235878,-2.47457185554549,-2.47456721633684,-2.47456249317495,
-2.47455768398931,-2.47455278693299,-2.47454780001297,-2.47454272104155,
-2.47453754790565,-2.4745322783669,-2.47345441286973,-2.47206186854742,
-2.46974466039954,-2.4554939036522,-2.45395997197966,-2.40802155766746,
-2.37916109038657,-2.37270998665603,-2.36999869161699,-2.3680368288707,
-2.36624523708514,-2.36338448544629,-2.35652334896222,-2.30318068000754,
-2.277470815958,-2.2662150159399,-2.26394582030786,-2.26269026979525,-2.26161909125403,
-2.26027082644707,-2.25764601760577,-2.24150091212544,-2.24101583413295,
-2.1912284482388,-2.16646318981933,-2.16051888163591,-2.15789537647367,
-2.15594889602381,-2.15413717743174,-2.15165157738876,-2.14535272088737,
-2.08663824047158,-2.06442962816323,-2.05412172347329,-2.05191024628017,
-2.05066726634226,-2.04959475679824,-2.04822924812027,-2.04605211190154,
-2.03448401034164,-2.03055853187892,-2.02328262038887,-2.00971921905664,
-1.97684352417414,-1.96029246488461,-1.94998765821279,-1.9467399055131,
-1.94466695264969,-1.94272645003395,-1.94018526537915,-1.93588969949699,
-1.90068511608129,-1.85146887356543,-1.84207165134789,-1.83992175857942,
-1.83869225630838,-1.8376177652025,-1.83623185099467,-1.83333112984071,
-1.80641914775787,-1.78860930819631,-1.74316008080986,-1.73677802729641,
-1.73407817692694,-1.73211818365603,-1.73032387676618,-1.72744914555655,
-1.72050450426299,-1.66826227906386,-1.64177462558227,-1.63032094645971,
-1.6280402111505,-1.62678205006324,-1.62571092940103,-1.62436564187795,
-1.62225506102581,-1.61176546417713,-1.60669564299256,-1.60640905281637,
-1.6050069692956,-1.59754472576318,-1.58574645830924,-1.5528830398556,-1.53634929533727,
-1.52605201131508,-1.52280489426815,-1.52073192976694,-1.51879112296061,
-1.5162491166074,-1.51195121246868,-1.47659221344915,-1.42743063198728,
-1.41811521441628,-1.41597103124672,-1.41474270437563,-1.4136678793923,
-1.41227973920362,-1.40936803809381,-1.37753527998185,-1.33437651320211,
-1.31573886100134,-1.31200614340079,-1.30960623516013,-1.30768946704697,
-1.30552191540457,-1.30184731996868,-1.28708441470362,-1.25997088998495),
 .UNSPECIFIED.);
#774=B_SPLINE_CURVE_WITH_KNOTS('',3,(#72748,#72749,#72750,#72751,#72752),
 .UNSPECIFIED.,.F.,.F.,(4,1,4),(82.6397395021165,82.9034253468356,82.9907454093913),
 .UNSPECIFIED.);
#775=B_SPLINE_CURVE_WITH_KNOTS('',3,(#72753,#72754,#72755,#72756,#72757,
#72758,#72759,#72760,#72761,#72762,#72763,#72764,#72765,#72766,#72767,#72768,
#72769,#72770,#72771,#72772,#72773,#72774,#72775,#72776,#72777,#72778,#72779,
#72780,#72781,#72782,#72783,#72784,#72785,#72786,#72787,#72788,#72789,#72790,
#72791,#72792,#72793,#72794,#72795,#72796,#72797,#72798,#72799,#72800,#72801,
#72802,#72803,#72804,#72805,#72806,#72807,#72808,#72809,#72810,#72811,#72812,
#72813,#72814,#72815,#72816,#72817,#72818,#72819,#72820,#72821,#72822,#72823,
#72824,#72825,#72826,#72827,#72828,#72829,#72830,#72831,#72832,#72833,#72834,
#72835,#72836,#72837,#72838,#72839,#72840,#72841,#72842,#72843,#72844,#72845,
#72846,#72847,#72848,#72849,#72850,#72851,#72852,#72853,#72854,#72855,#72856,
#72857,#72858,#72859,#72860,#72861,#72862,#72863,#72864,#72865,#72866,#72867,
#72868,#72869,#72870,#72871,#72872,#72873,#72874,#72875,#72876,#72877,#72878,
#72879,#72880,#72881,#72882,#72883,#72884,#72885,#72886,#72887,#72888,#72889,
#72890,#72891,#72892,#72893,#72894,#72895,#72896,#72897,#72898,#72899,#72900,
#72901,#72902,#72903,#72904,#72905,#72906,#72907,#72908,#72909,#72910,#72911,
#72912,#72913,#72914,#72915,#72916,#72917,#72918,#72919,#72920,#72921,#72922,
#72923,#72924,#72925,#72926,#72927,#72928,#72929,#72930,#72931,#72932,#72933,
#72934,#72935,#72936,#72937,#72938,#72939,#72940,#72941,#72942,#72943,#72944,
#72945,#72946,#72947,#72948,#72949,#72950,#72951,#72952,#72953,#72954,#72955,
#72956,#72957,#72958,#72959,#72960,#72961,#72962,#72963,#72964,#72965,#72966,
#72967,#72968,#72969,#72970,#72971,#72972,#72973,#72974,#72975,#72976,#72977,
#72978,#72979,#72980,#72981,#72982,#72983,#72984,#72985,#72986,#72987,#72988,
#72989,#72990,#72991,#72992,#72993,#72994,#72995,#72996,#72997,#72998,#72999,
#73000,#73001,#73002,#73003,#73004,#73005,#73006,#73007,#73008,#73009,#73010),
 .UNSPECIFIED.,.F.,.F.,(4,2,2,2,2,2,2,2,2,2,2,2,2,2,2,2,2,2,2,2,2,2,2,2,
2,2,2,2,2,2,2,2,2,2,2,2,2,2,2,2,2,2,2,2,2,2,2,2,2,2,2,2,2,2,2,2,2,2,2,2,
2,2,2,2,2,2,2,2,2,2,2,2,2,2,2,2,2,2,2,2,2,2,2,2,2,2,2,2,2,2,2,2,2,2,2,2,
2,2,2,2,2,2,2,2,2,2,2,2,2,2,2,2,2,2,2,2,2,2,2,2,2,2,2,2,2,2,2,2,4),(-2.66768858982521,
-2.61548896877153,-2.59709218284674,-2.58597251558751,-2.58263451317238,
-2.58054173678217,-2.57860857796354,-2.5761135948932,-2.57197620698229,
-2.54431964197868,-2.50203657869528,-2.48608860941616,-2.48055584025264,
-2.47791674022811,-2.47580170224508,-2.47457852674913,-2.47457497998066,
-2.47457141961672,-2.47456784565589,-2.47456425770073,-2.47456065578851,
-2.47455676068287,-2.47455279767257,-2.47454876538423,-2.4745446621522,
-2.47454048653611,-2.47453623699223,-2.47453191195419,-2.47452750977546,
-2.47452302865531,-2.47451846685654,-2.47349995987621,-2.47213831295872,
-2.4693606005064,-2.44976951333447,-2.40678477004586,-2.37604589982498,
-2.37160172333146,-2.36926829660271,-2.36735663298897,-2.36514152603537,
-2.36135107466242,-2.34671264791226,-2.33445992859165,-2.2940883402603,
-2.27526162494784,-2.26597271472751,-2.26383073347549,-2.26260303948821,
-2.26152835828382,-2.26013986258116,-2.25722550529324,-2.22720436744997,
-2.22134525855173,-2.18858927941237,-2.16604120359468,-2.16038964584546,
-2.15781898892924,-2.15588087587657,-2.15405439840896,-2.15151263101193,
-2.14487102325656,-2.08908347801888,-2.06501753820829,-2.05419381562661,
-2.05195004850705,-2.05069996338546,-2.04962816109695,-2.04827233538406,
-2.04612717251834,-2.03509364883462,-1.98380446409605,-1.95516390243856,
-1.94873875176907,-1.94603172128124,-1.94407053306687,-1.94227789866082,
-1.93941187568713,-1.93251940555216,-1.87956931497458,-1.85358275109322,
-1.84225593726981,-1.83998254241669,-1.83872602773826,-1.83765485189969,
-1.83630764114471,-1.83368797587197,-1.8176741187007,-1.81224529340355,
-1.79776915784436,-1.76488248766917,-1.74831911116621,-1.73800862446994,
-1.73476013975599,-1.73268697391084,-1.73074645051109,-1.72820549631391,
-1.72391089752837,-1.68879247073889,-1.63986091691466,-1.63013049875607,
-1.62795721093769,-1.62672252855143,-1.6256487838211,-1.62427073719501,
-1.62205244279046,-1.60975260750496,-1.60659787281006,-1.60639522129257,
-1.60500788913289,-1.59754454953592,-1.58574638597926,-1.55288297089003,
-1.5363492285818,-1.52605194581472,-1.52280482910815,-1.52073186481134,
-1.51879105818772,-1.51624905206128,-1.51195114827854,-1.47659214975019,
-1.427430573787,-1.41811515732466,-1.41597097437513,-1.41474264762363,-1.4136678227414,
-1.41227968268057,-1.40936798182881,-1.40856908540218),.UNSPECIFIED.);
#776=B_SPLINE_CURVE_WITH_KNOTS('',3,(#73012,#73013,#73014,#73015,#73016,
#73017,#73018,#73019,#73020,#73021,#73022,#73023,#73024,#73025,#73026,#73027,
#73028,#73029,#73030,#73031,#73032,#73033,#73034,#73035,#73036,#73037,#73038,
#73039,#73040,#73041,#73042,#73043,#73044,#73045,#73046,#73047,#73048,#73049,
#73050,#73051,#73052,#73053,#73054,#73055,#73056,#73057,#73058,#73059,#73060,
#73061,#73062,#73063,#73064,#73065,#73066,#73067,#73068,#73069,#73070,#73071,
#73072,#73073,#73074,#73075,#73076,#73077,#73078,#73079,#73080,#73081,#73082,
#73083,#73084,#73085,#73086,#73087,#73088,#73089,#73090,#73091,#73092,#73093,
#73094,#73095,#73096,#73097,#73098,#73099,#73100,#73101,#73102,#73103,#73104,
#73105,#73106,#73107,#73108,#73109,#73110,#73111,#73112,#73113,#73114,#73115,
#73116,#73117,#73118,#73119,#73120,#73121,#73122,#73123,#73124,#73125,#73126,
#73127,#73128,#73129,#73130,#73131,#73132,#73133,#73134,#73135,#73136,#73137,
#73138,#73139,#73140,#73141,#73142,#73143,#73144,#73145,#73146,#73147,#73148,
#73149,#73150,#73151,#73152,#73153,#73154,#73155,#73156,#73157,#73158,#73159,
#73160,#73161,#73162,#73163,#73164,#73165,#73166,#73167,#73168,#73169,#73170,
#73171,#73172,#73173,#73174,#73175,#73176,#73177,#73178,#73179,#73180,#73181,
#73182,#73183,#73184,#73185,#73186,#73187,#73188,#73189,#73190,#73191,#73192,
#73193,#73194,#73195,#73196,#73197,#73198,#73199,#73200,#73201,#73202,#73203,
#73204,#73205,#73206,#73207,#73208,#73209,#73210,#73211,#73212,#73213,#73214,
#73215,#73216,#73217,#73218,#73219,#73220,#73221,#73222,#73223,#73224,#73225,
#73226,#73227),.UNSPECIFIED.,.F.,.F.,(4,2,2,2,2,2,2,2,2,2,2,2,2,2,2,2,2,
2,2,2,2,2,2,2,2,2,2,2,2,2,2,2,2,2,2,2,2,2,2,2,2,2,2,2,2,2,2,2,2,2,2,2,2,
2,2,2,2,2,2,2,2,2,2,2,2,2,2,2,2,2,2,2,2,2,2,2,2,2,2,2,2,2,2,2,2,2,2,2,2,
2,2,2,2,2,2,2,2,2,2,2,2,2,2,2,2,2,2,4),(-1.25997088998495,-1.25915938594851,
-1.20936246129004,-1.20515951081736,-1.20349953697922,-1.20248974489613,
-1.20138550293452,-1.19981051724376,-1.19583461291313,-1.17602195020207,
-1.14710915924182,-1.10479023230581,-1.10049511966369,-1.09795388032023,
-1.09601313909686,-1.09393973957955,-1.09069088550478,-1.08037911476509,
-1.0638158766874,-1.03095510860562,-1.01703048962702,-1.01060094149894,
-0.995017859170259,-0.992416308889875,-0.991072921165533,-0.990001879297503,
-0.988742148630458,-0.986454303225226,-0.974875759619038,-0.947884438765955,
-0.896303807819882,-0.889312882965154,-0.886430439299655,-0.884634679239556,
-0.882675788452561,-0.879982350025813,-0.873638319236514,-0.845679922156646,
-0.799187143952254,-0.783069530515761,-0.780442292428072,-0.779093389562779,
-0.778022023285564,-0.776766628080356,-0.774498653501712,-0.763268518759134,
-0.737658607207535,-0.684115422820024,-0.677266049977641,-0.674406981219692,
-0.672615510694201,-0.67065303473273,-0.667939512583055,-0.661476520998392,
-0.607432539657972,-0.57135384080706,-0.568495481477209,-0.567117807054397,
-0.566044085688787,-0.564809137742537,-0.562634670186238,-0.552887583070529,
-0.503943804097238,-0.468812369254383,-0.464519859198177,-0.461979550208044,
-0.460039168375182,-0.457965812272562,-0.454716314930514,-0.444396501120506,
-0.427814631244484,-0.371116881744046,-0.358713447202724,-0.356489604077167,
-0.355109878850799,-0.354035970281442,-0.352802397213448,-0.350634140673739,
-0.340976935671784,-0.291957487243451,-0.256812038695503,-0.252513704361133,
-0.249971722796989,-0.248031084683539,-0.246240436043974,-0.243303027853584,
-0.235328349705132,-0.223524277204574,-0.190998983152449,-0.15007844644583,
-0.145387645993221,-0.143651116808162,-0.14262662328381,-0.141533912165226,
-0.140020750544341,-0.136420730740827,-0.0985295544978921,-0.075735779521925,
-0.0634020308221991,-0.0604357883634491,-0.0436144641611536,-0.0399995481703897,
-0.0376361127493614,-0.0357225149470006,-0.0339209956216892,-0.0317709078565799,
-0.0286342760631504,-0.000628476376618018),.UNSPECIFIED.);
#777=B_SPLINE_CURVE_WITH_KNOTS('',3,(#73228,#73229,#73230,#73231,#73232,
#73233,#73234,#73235,#73236,#73237,#73238,#73239,#73240,#73241,#73242,#73243,
#73244,#73245),.UNSPECIFIED.,.F.,.F.,(4,2,2,2,2,2,2,2,4),(-2.66749886584903,
-2.62118884059196,-2.60358532551492,-2.5998480387605,-2.59831158971457,
-2.59721449148509,-2.5961956497179,-2.59448907267751,-2.59335004581682),
 .UNSPECIFIED.);
#778=B_SPLINE_CURVE_WITH_KNOTS('',3,(#73251,#73252,#73253,#73254,#73255,
#73256,#73257,#73258,#73259,#73260,#73261,#73262,#73263),.UNSPECIFIED.,
 .F.,.F.,(4,3,3,3,4),(76.3573194796184,76.4589088025925,76.5605127982575,
76.6622238139045,76.707559910557),.UNSPECIFIED.);
#779=B_SPLINE_CURVE_WITH_KNOTS('',3,(#73264,#73265,#73266,#73267,#73268,
#73269,#73270,#73271,#73272,#73273),.UNSPECIFIED.,.F.,.F.,(4,1,1,1,1,1,
1,4),(76.7075601022117,76.9104066470643,77.9092430970262,78.9080795469881,
79.90691599695,80.9057524469119,81.9045888968737,82.6397395021165),
 .UNSPECIFIED.);
#780=B_SPLINE_CURVE_WITH_KNOTS('',3,(#73274,#73275,#73276,#73277,#73278,
#73279,#73280,#73281,#73282,#73283,#73284,#73285,#73286,#73287,#73288,#73289,
#73290,#73291,#73292,#73293,#73294,#73295,#73296,#73297,#73298,#73299,#73300,
#73301,#73302,#73303,#73304,#73305,#73306,#73307,#73308,#73309,#73310,#73311,
#73312,#73313,#73314,#73315,#73316,#73317,#73318,#73319,#73320,#73321,#73322,
#73323,#73324,#73325,#73326,#73327,#73328,#73329,#73330,#73331,#73332,#73333,
#73334,#73335,#73336,#73337,#73338,#73339,#73340,#73341,#73342,#73343,#73344,
#73345,#73346,#73347,#73348,#73349,#73350,#73351,#73352,#73353,#73354,#73355,
#73356,#73357,#73358,#73359,#73360,#73361,#73362,#73363,#73364,#73365,#73366,
#73367,#73368,#73369,#73370,#73371,#73372,#73373,#73374,#73375,#73376,#73377,
#73378,#73379,#73380,#73381,#73382,#73383,#73384,#73385,#73386,#73387,#73388,
#73389,#73390,#73391,#73392,#73393,#73394,#73395,#73396,#73397,#73398,#73399,
#73400,#73401,#73402,#73403,#73404,#73405,#73406,#73407,#73408,#73409,#73410,
#73411,#73412,#73413,#73414,#73415,#73416,#73417,#73418,#73419,#73420,#73421,
#73422,#73423,#73424,#73425,#73426,#73427,#73428,#73429,#73430,#73431,#73432,
#73433,#73434,#73435,#73436,#73437,#73438,#73439,#73440,#73441,#73442,#73443,
#73444,#73445,#73446,#73447,#73448,#73449,#73450,#73451,#73452,#73453,#73454,
#73455,#73456,#73457,#73458,#73459,#73460,#73461,#73462,#73463,#73464,#73465,
#73466,#73467,#73468,#73469,#73470,#73471,#73472,#73473,#73474,#73475,#73476,
#73477,#73478,#73479,#73480,#73481,#73482,#73483,#73484,#73485,#73486,#73487,
#73488,#73489,#73490,#73491,#73492,#73493,#73494,#73495,#73496,#73497,#73498,
#73499,#73500,#73501,#73502,#73503,#73504,#73505,#73506,#73507,#73508,#73509),
 .UNSPECIFIED.,.F.,.F.,(4,2,2,2,2,2,2,2,2,2,2,2,2,2,2,2,2,2,2,2,2,2,2,2,
2,2,2,2,2,2,2,2,2,2,2,2,2,2,2,2,2,2,2,2,2,2,2,2,2,2,2,2,2,2,2,2,2,2,2,2,
2,2,2,2,2,2,2,2,2,2,2,2,2,2,2,2,2,2,2,2,2,2,2,2,2,2,2,2,2,2,2,2,2,2,2,2,
2,2,2,2,2,2,2,2,2,2,2,2,2,2,2,2,2,2,2,2,2,4),(-2.59335004581682,-2.58999661647289,
-2.54298822566556,-2.52282531450821,-2.50695145909145,-2.50030351558134,
-2.49524072965445,-2.49278360397924,-2.49085430630762,-2.48900664979301,
-2.48585214961438,-2.47714077652947,-2.47621720966657,-2.42660199449724,
-2.40064010349671,-2.38931836114964,-2.38704484075098,-2.38578810308318,
-2.38471664392004,-2.38336895814841,-2.38074802022203,-2.36471991080766,
-2.35646656727578,-2.31512128777579,-2.29646839836423,-2.2852377555109,
-2.28188729080691,-2.27979135151281,-2.27785842862949,-2.27536816262005,
-2.27124813843114,-2.24430743096339,-2.20161635166961,-2.18540412607491,
-2.17698169006088,-2.17490542676618,-2.17369204246962,-2.17261418945241,
-2.17122414614609,-2.16891628770687,-2.15484859550471,-2.14363434223291,
-2.10759082339872,-2.07836174403861,-2.07186583929587,-2.06914637507462,
-2.06718244016351,-2.0653915856908,-2.06253770342873,-2.05572235948569,
-2.00176933962491,-1.97645424138811,-1.96529851669718,-1.9630344988653,
-1.96177977212936,-1.96070805213172,-1.95935751814658,-1.95672360049277,
-1.94037023846529,-1.93130268342654,-1.89233486680948,-1.86585535645503,
-1.85969246019393,-1.85702977428294,-1.85507592961925,-1.85327266367671,
-1.85035119746512,-1.84312955644879,-1.79876310021537,-1.78472961336681,
-1.76327504185664,-1.75318360347803,-1.75098563009592,-1.74974532528916,
-1.74867202217588,-1.74730147530282,-1.74510859862459,-1.73333817430004,
-1.72962679302802,-1.72236561755901,-1.67901009945593,-1.66042269314622,
-1.64921988552873,-1.64587222371128,-1.64377680994162,-1.64184353799485,
-1.63935165754725,-1.63522644470455,-1.60809058835119,-1.56616639778275,
-1.54954738105999,-1.54098479617681,-1.53889724539177,-1.53768130649548,
-1.53660391444603,-1.53521798987499,-1.53292428426228,-1.51915035003429,
-1.50784475920294,-1.46844818184545,-1.4418753879567,-1.43570087708518,
-1.43303616922358,-1.43108196856404,-1.42927916587146,-1.4263602192889,
-1.41915355534996,-1.37307257018466,-1.33396208825774,-1.33297752449863,
-1.32826981195437,-1.32653033376173,-1.32550500699202,-1.32441217670042,
-1.32290010594739,-1.31930847052064,-1.28016891975437,-1.25968440179264),
 .UNSPECIFIED.);
#781=B_SPLINE_CURVE_WITH_KNOTS('',3,(#73515,#73516,#73517,#73518,#73519,
#73520,#73521,#73522,#73523,#73524,#73525,#73526,#73527,#73528,#73529,#73530,
#73531,#73532),.UNSPECIFIED.,.F.,.F.,(4,2,2,2,2,2,2,2,4),(-0.0749304253432432,
-0.0455284962237961,-0.0267278979708963,-0.0187639971196157,-0.00802108746917657,
-0.00466632884064646,-0.00258130080575418,-0.00128118374794539,-0.000628942230927431),
 .UNSPECIFIED.);
#782=B_SPLINE_CURVE_WITH_KNOTS('',3,(#73533,#73534,#73535,#73536,#73537,
#73538,#73539,#73540,#73541,#73542,#73543,#73544,#73545,#73546,#73547,#73548,
#73549,#73550,#73551,#73552,#73553,#73554,#73555,#73556,#73557,#73558,#73559,
#73560,#73561,#73562,#73563,#73564,#73565,#73566,#73567,#73568,#73569,#73570,
#73571,#73572,#73573,#73574,#73575,#73576,#73577,#73578,#73579,#73580,#73581,
#73582,#73583,#73584,#73585,#73586,#73587,#73588,#73589,#73590,#73591,#73592,
#73593,#73594,#73595,#73596,#73597,#73598,#73599,#73600,#73601,#73602,#73603,
#73604,#73605,#73606,#73607,#73608,#73609,#73610,#73611,#73612,#73613,#73614,
#73615,#73616,#73617,#73618,#73619,#73620,#73621,#73622,#73623,#73624,#73625,
#73626,#73627,#73628,#73629,#73630,#73631,#73632,#73633,#73634,#73635,#73636,
#73637,#73638,#73639,#73640,#73641,#73642,#73643,#73644,#73645,#73646,#73647,
#73648,#73649,#73650,#73651,#73652,#73653,#73654,#73655,#73656,#73657,#73658,
#73659,#73660,#73661,#73662,#73663,#73664,#73665,#73666,#73667,#73668,#73669,
#73670,#73671,#73672,#73673,#73674,#73675,#73676,#73677,#73678,#73679,#73680,
#73681,#73682,#73683,#73684,#73685,#73686,#73687,#73688,#73689,#73690,#73691,
#73692,#73693,#73694,#73695,#73696,#73697,#73698,#73699,#73700,#73701,#73702,
#73703,#73704,#73705,#73706,#73707,#73708,#73709,#73710,#73711,#73712,#73713),
 .UNSPECIFIED.,.F.,.F.,(4,3,3,3,3,3,3,3,3,3,3,3,3,3,3,3,3,3,3,3,3,3,3,3,
3,3,3,3,3,3,3,3,3,3,3,3,3,3,3,3,3,3,3,3,3,3,3,3,3,3,3,3,3,3,3,3,3,3,3,3,
4),(70.4243747954073,70.5325790413758,70.6410991164239,70.7497863837817,
70.8587740112793,70.9173879472931,71.0207826843411,71.1240239664562,71.2271439318486,
71.3301985000576,71.4332217084154,71.5362475510879,71.639380317866,71.7425694092759,
71.8459414026576,71.916224397255,72.0196191343029,72.1228604164179,72.2259803818102,
72.3290349500191,72.4320581583768,72.5350840010492,72.6382167678273,72.7414058592371,
72.8447778526187,72.9150608472168,73.0184555842647,73.1216968663797,73.224816831772,
73.3278713999809,73.4308946083386,73.5339204510111,73.6370532177892,73.740242309199,
73.8436143025806,73.9138972971787,74.0172920342267,74.1205333163417,74.223653281734,
74.326707849943,74.4297310583007,74.5327569009732,74.6358896677513,74.7390787591612,
74.8424507525428,74.9127337471406,75.0161284841886,75.1193697663036,75.2224897316959,
75.3255442999048,75.4285675082626,75.531593350935,75.6347261177131,75.7379152091229,
75.8412872025045,75.9115701971025,76.0134810050385,76.1152211478776,76.2168630906285,
76.3184433457388,76.3573194796184),.UNSPECIFIED.);
#783=B_SPLINE_CURVE_WITH_KNOTS('',3,(#73715,#73716,#73717,#73718,#73719,
#73720,#73721,#73722,#73723,#73724,#73725,#73726,#73727,#73728,#73729,#73730,
#73731,#73732,#73733,#73734,#73735,#73736,#73737,#73738,#73739,#73740,#73741,
#73742,#73743,#73744,#73745,#73746,#73747,#73748,#73749,#73750,#73751,#73752,
#73753,#73754,#73755,#73756,#73757,#73758,#73759,#73760,#73761,#73762,#73763,
#73764,#73765,#73766,#73767,#73768,#73769,#73770,#73771,#73772,#73773,#73774,
#73775,#73776,#73777,#73778,#73779,#73780,#73781,#73782,#73783,#73784,#73785,
#73786,#73787,#73788,#73789,#73790,#73791,#73792,#73793,#73794,#73795,#73796,
#73797,#73798,#73799,#73800,#73801,#73802,#73803,#73804,#73805,#73806,#73807,
#73808,#73809,#73810,#73811,#73812,#73813,#73814,#73815,#73816,#73817,#73818,
#73819,#73820,#73821,#73822,#73823,#73824,#73825,#73826,#73827,#73828,#73829,
#73830,#73831,#73832,#73833,#73834,#73835,#73836,#73837,#73838,#73839,#73840,
#73841,#73842,#73843,#73844,#73845,#73846,#73847,#73848,#73849,#73850,#73851,
#73852,#73853,#73854,#73855,#73856,#73857,#73858,#73859,#73860,#73861,#73862,
#73863,#73864,#73865,#73866,#73867,#73868,#73869,#73870,#73871,#73872,#73873,
#73874,#73875,#73876,#73877,#73878,#73879,#73880,#73881,#73882,#73883,#73884,
#73885,#73886,#73887,#73888,#73889,#73890,#73891,#73892,#73893,#73894,#73895,
#73896,#73897,#73898,#73899,#73900,#73901,#73902,#73903,#73904,#73905,#73906,
#73907,#73908,#73909,#73910,#73911,#73912,#73913,#73914,#73915,#73916,#73917,
#73918,#73919,#73920,#73921,#73922,#73923,#73924,#73925,#73926,#73927,#73928,
#73929,#73930),.UNSPECIFIED.,.F.,.F.,(4,2,2,2,2,2,2,2,2,2,2,2,2,2,2,2,2,
2,2,2,2,2,2,2,2,2,2,2,2,2,2,2,2,2,2,2,2,2,2,2,2,2,2,2,2,2,2,2,2,2,2,2,2,
2,2,2,2,2,2,2,2,2,2,2,2,2,2,2,2,2,2,2,2,2,2,2,2,2,2,2,2,2,2,2,2,2,2,2,2,
2,2,2,2,2,2,2,2,2,2,2,2,2,2,2,2,2,2,4),(-1.25968440179264,-1.23134354359258,
-1.22421237516867,-1.22130613530729,-1.21950569996339,-1.21754974618457,
-1.21487487073439,-1.20864141476093,-1.18159524773247,-1.14086775040501,
-1.11820863565655,-1.11535573719631,-1.11397894883129,-1.11290509685899,
-1.11166907107165,-1.10949048549418,-1.09968816714513,-1.05077794022017,
-1.0156573334309,-1.01136167951513,-1.00882016350117,-1.00687923608233,
-1.00480566197672,-1.00155658514622,-0.991244535768014,-0.974681257565122,
-0.941818689315611,-0.928011237409794,-0.921314019760237,-0.905865110191607,
-0.903497154921353,-0.902089561422103,-0.901009403711653,-0.899805960922281,
-0.897774187092332,-0.889884288291235,-0.875167986218626,-0.846104074711493,
-0.803698149660333,-0.799404686669405,-0.796863862765149,-0.794923115869781,
-0.792849397085583,-0.789599388560396,-0.779278434431453,-0.762695192216084,
-0.729816909009761,-0.71451639446695,-0.709793784952005,-0.69394156356986,
-0.6913287511807,-0.689982894230297,-0.688911650363044,-0.687653733401105,
-0.685374422218113,-0.673948886331171,-0.647572501794949,-0.59512229006198,
-0.588188792919766,-0.585315749203526,-0.583521642465524,-0.581561190123421,
-0.578859461115646,-0.572467090465569,-0.526046462190321,-0.484947958096599,
-0.480263100775048,-0.478527318893239,-0.477502868156652,-0.476409864053683,
-0.474895743400699,-0.471290883635746,-0.432950265486838,-0.383317351113001,
-0.376221655519629,-0.373321731023507,-0.371522738030721,-0.36956639584249,
-0.366887460089059,-0.360806569983863,-0.352445732563901,-0.301551240269501,
-0.27031324179841,-0.267401274645498,-0.266013097821487,-0.264938282186225,
-0.263710017433473,-0.261566048832606,-0.252414968969124,-0.203666437397408,
-0.167704290380167,-0.162982356583487,-0.160559558302476,-0.158640677010409,
-0.156487803395795,-0.154258048298956,-0.146612096948347,-0.121083045479512,
-0.100337617846573,-0.0610229399657464,-0.0562870051492831,-0.0545435818946793,
-0.0535177060778159,-0.0524257934789496,-0.0509174405909417,-0.0492296220639371,
-0.0462824118400645,-0.00062912028025528),.UNSPECIFIED.);
#784=B_SPLINE_CURVE_WITH_KNOTS('',3,(#73931,#73932,#73933,#73934,#73935,
#73936,#73937,#73938,#73939,#73940,#73941,#73942,#73943),.UNSPECIFIED.,
 .F.,.F.,(4,3,3,3,4),(-66.6728921052185,-66.5709585796832,-66.4690950147654,
-66.3672509448922,-66.3228588019918),.UNSPECIFIED.);
#785=B_SPLINE_CURVE_WITH_KNOTS('',3,(#73948,#73949,#73950,#73951,#73952,
#73953,#73954,#73955,#73956,#73957,#73958,#73959,#73960,#73961,#73962,#73963,
#73964,#73965,#73966,#73967,#73968,#73969,#73970,#73971,#73972,#73973,#73974,
#73975,#73976,#73977,#73978,#73979,#73980,#73981,#73982,#73983,#73984,#73985,
#73986,#73987,#73988,#73989,#73990,#73991,#73992,#73993,#73994,#73995,#73996,
#73997,#73998,#73999,#74000,#74001,#74002,#74003,#74004,#74005,#74006,#74007,
#74008,#74009,#74010,#74011,#74012,#74013,#74014,#74015,#74016,#74017,#74018,
#74019,#74020,#74021,#74022,#74023,#74024,#74025,#74026,#74027,#74028,#74029,
#74030,#74031,#74032,#74033,#74034,#74035,#74036,#74037,#74038,#74039,#74040,
#74041,#74042,#74043,#74044,#74045,#74046,#74047,#74048,#74049,#74050,#74051,
#74052,#74053,#74054,#74055,#74056,#74057,#74058,#74059,#74060,#74061,#74062,
#74063,#74064,#74065,#74066,#74067,#74068,#74069,#74070,#74071,#74072,#74073,
#74074,#74075,#74076,#74077,#74078,#74079,#74080,#74081,#74082,#74083,#74084,
#74085,#74086,#74087,#74088,#74089,#74090,#74091,#74092,#74093,#74094,#74095,
#74096,#74097,#74098,#74099,#74100,#74101,#74102,#74103,#74104,#74105,#74106,
#74107,#74108,#74109,#74110,#74111,#74112,#74113,#74114,#74115,#74116,#74117,
#74118,#74119,#74120,#74121,#74122,#74123,#74124,#74125,#74126,#74127,#74128,
#74129,#74130,#74131,#74132,#74133,#74134,#74135,#74136,#74137,#74138,#74139,
#74140,#74141,#74142,#74143,#74144,#74145,#74146,#74147,#74148,#74149,#74150,
#74151,#74152,#74153,#74154,#74155,#74156,#74157,#74158,#74159,#74160,#74161,
#74162,#74163,#74164,#74165,#74166,#74167,#74168,#74169,#74170,#74171,#74172,
#74173,#74174,#74175,#74176,#74177,#74178,#74179,#74180,#74181,#74182,#74183),
 .UNSPECIFIED.,.F.,.F.,(4,2,2,2,2,2,2,2,2,2,2,2,2,2,2,2,2,2,2,2,2,2,2,2,
2,2,2,2,2,2,2,2,2,2,2,2,2,2,2,2,2,2,2,2,2,2,2,2,2,2,2,2,2,2,2,2,2,2,2,2,
2,2,2,2,2,2,2,2,2,2,2,2,2,2,2,2,2,2,2,2,2,2,2,2,2,2,2,2,2,2,2,2,2,2,2,2,
2,2,2,2,2,2,2,2,2,2,2,2,2,2,2,2,2,2,2,2,2,4),(-1.40858075324139,-1.3954320310824,
-1.38403044609259,-1.38175218761962,-1.38049433958623,-1.37942284788281,
-1.37807628373716,-1.37546093967725,-1.35953982828857,-1.3550374675103,
-1.33447375915959,-1.28611804330527,-1.2789688130659,-1.27605948095026,
-1.27425842721691,-1.27230282560658,-1.26963027500151,-1.2634106407658,
-1.236477491613,-1.19595077061155,-1.17295835890062,-1.17010289559586,-1.16872557241452,
-1.16765163385077,-1.16641588170656,-1.16423867208337,-1.1544573691123,
-1.10552726911894,-1.07039940615101,-1.06610351061807,-1.06356187536306,
-1.06162087053721,-1.05954722697486,-1.05629806895955,-1.045985994997,-1.02942289900999,
-0.996559755773456,-0.982817040336085,-0.975966154357702,-0.975652096740871,
-0.970071493947574,-0.960066604665169,-0.957987944541318,-0.956652334414198,
-0.955581600488022,-0.95431533213327,-0.951997722631066,-0.939874527391814,
-0.887010946290296,-0.858184668381248,-0.85401554228252,-0.851511002737233,
-0.849576079450493,-0.847486992237177,-0.844166926328647,-0.833217602457786,
-0.815218071557374,-0.764880679873219,-0.748636138557531,-0.746006908141442,
-0.744657497923189,-0.743585998854998,-0.742330760681044,-0.740063861275224,
-0.728855049170755,-0.703329670730521,-0.649654556879947,-0.64281484722695,
-0.639957196981804,-0.638165854861379,-0.636202906072923,-0.63348760102407,
-0.627014974625186,-0.572643457020699,-0.565705913317623,-0.536988933091167,
-0.534076816790993,-0.53268857431109,-0.53161371034783,-0.530385393173036,
-0.528241339642794,-0.518928532966178,-0.469757761828656,-0.434365043220982,
-0.430066107429614,-0.427523821151675,-0.425582979749055,-0.423510150961256,
-0.42026360554307,-0.409971071037893,-0.393450040703956,-0.360625201356664,
-0.350841379626458,-0.32499280592247,-0.322101634848752,-0.320717556899922,
-0.319643221873447,-0.318412484745028,-0.316257085837481,-0.306783343152919,
-0.257606400046225,-0.222412842168993,-0.217734027536337,-0.215348525553729,
-0.213485530932822,-0.211693643003537,-0.208571161773771,-0.199305098970657,
-0.18498357052622,-0.124681947776451,-0.11228550953053,-0.110062031709171,
-0.108682412250948,-0.1076085081102,-0.106374852361822,-0.104206241556676,
-0.0945440565291435,-0.0749304253432432),.UNSPECIFIED.);
#786=B_SPLINE_CURVE_WITH_KNOTS('',3,(#74185,#74186,#74187,#74188,#74189,
#74190,#74191,#74192,#74193,#74194,#74195,#74196,#74197,#74198,#74199,#74200,
#74201,#74202,#74203,#74204,#74205,#74206,#74207,#74208,#74209,#74210,#74211,
#74212,#74213,#74214,#74215,#74216,#74217,#74218,#74219,#74220,#74221,#74222,
#74223,#74224,#74225,#74226,#74227,#74228,#74229,#74230,#74231,#74232,#74233,
#74234,#74235,#74236,#74237,#74238,#74239,#74240,#74241,#74242,#74243,#74244,
#74245,#74246,#74247,#74248,#74249,#74250,#74251,#74252,#74253,#74254,#74255,
#74256,#74257,#74258,#74259,#74260,#74261,#74262,#74263,#74264,#74265,#74266,
#74267,#74268,#74269,#74270,#74271,#74272,#74273,#74274,#74275,#74276,#74277,
#74278,#74279,#74280,#74281,#74282,#74283,#74284,#74285,#74286,#74287,#74288,
#74289,#74290,#74291,#74292,#74293,#74294,#74295,#74296,#74297,#74298,#74299,
#74300,#74301,#74302,#74303,#74304,#74305,#74306,#74307,#74308,#74309,#74310,
#74311,#74312,#74313,#74314,#74315,#74316,#74317,#74318,#74319,#74320,#74321,
#74322,#74323,#74324,#74325,#74326,#74327,#74328,#74329,#74330,#74331,#74332,
#74333,#74334,#74335,#74336,#74337,#74338,#74339,#74340,#74341,#74342,#74343,
#74344,#74345,#74346,#74347,#74348,#74349,#74350,#74351,#74352,#74353,#74354,
#74355,#74356,#74357,#74358,#74359,#74360,#74361,#74362),.UNSPECIFIED.,
 .F.,.F.,(4,3,3,3,3,3,3,3,3,3,3,3,3,3,3,3,3,3,3,3,3,3,3,3,3,3,3,3,3,3,3,
3,3,3,3,3,3,3,3,3,3,3,3,3,3,3,3,3,3,3,3,3,3,3,3,3,3,3,3,4),(-66.3228588019918,
-66.2209269508808,-66.1189508703786,-66.0167874549306,-65.9232056974837,
-65.8198109604357,-65.7165696783206,-65.6134497129283,-65.5103951447194,
-65.4073719363618,-65.3043460936894,-65.2012133269113,-65.0980242355016,
-64.99465224212,-64.9243692475218,-64.820974510474,-64.7177332283591,-64.6146132629669,
-64.5115586947579,-64.4085354864001,-64.3055096437278,-64.2023768769497,
-64.09918778554,-63.9958157921584,-63.92553279756,-63.8221380605121,-63.7188967783972,
-63.6157768130049,-63.512722244796,-63.4096990364381,-63.3066731937657,
-63.2035404269877,-63.1003513355779,-62.9969793421963,-62.9266963475981,
-62.8233016105501,-62.7200603284351,-62.6169403630427,-62.5138857948337,
-62.4108625864758,-62.3078367438028,-62.2047039770247,-62.101514885615,
-61.9981428922333,-61.9278598976362,-61.8244651605883,-61.721223878473,
-61.6181039130809,-61.515049344872,-61.4120261365142,-61.3090002938415,
-61.2058675270636,-61.1026784356539,-60.9993064422722,-60.9290234476744,
-60.8220651862381,-60.7139755891883,-60.6074364851713,-60.4985716416051,
-60.3897067980389),.UNSPECIFIED.);
#787=B_SPLINE_CURVE_WITH_KNOTS('',3,(#74363,#74364,#74365,#74366),
 .UNSPECIFIED.,.F.,.F.,(4,4),(-60.3897037700897,-60.0402340406592),
 .UNSPECIFIED.);
#788=B_SPLINE_CURVE_WITH_KNOTS('',3,(#74372,#74373,#74374,#74375,#74376,
#74377),.UNSPECIFIED.,.F.,.F.,(4,2,4),(-0.0750411156564984,-0.0537578376115912,
-0.000629603145374127),.UNSPECIFIED.);
#789=B_SPLINE_CURVE_WITH_KNOTS('',3,(#74378,#74379,#74380,#74381,#74382,
#74383,#74384,#74385,#74386,#74387,#74388,#74389,#74390,#74391,#74392,#74393,
#74394,#74395,#74396,#74397,#74398,#74399,#74400,#74401,#74402,#74403,#74404,
#74405,#74406,#74407,#74408,#74409,#74410,#74411,#74412,#74413,#74414,#74415,
#74416,#74417,#74418,#74419,#74420,#74421,#74422,#74423,#74424,#74425,#74426,
#74427,#74428,#74429,#74430,#74431,#74432,#74433,#74434,#74435,#74436,#74437,
#74438,#74439,#74440,#74441,#74442,#74443,#74444,#74445,#74446,#74447,#74448,
#74449,#74450,#74451,#74452,#74453,#74454,#74455,#74456,#74457,#74458,#74459,
#74460,#74461,#74462,#74463,#74464,#74465,#74466,#74467,#74468,#74469,#74470,
#74471,#74472,#74473,#74474,#74475,#74476,#74477,#74478,#74479,#74480,#74481,
#74482,#74483,#74484,#74485,#74486,#74487,#74488,#74489,#74490,#74491,#74492,
#74493,#74494,#74495,#74496,#74497,#74498,#74499,#74500,#74501,#74502,#74503,
#74504,#74505,#74506,#74507,#74508,#74509,#74510,#74511,#74512,#74513,#74514,
#74515,#74516,#74517,#74518,#74519,#74520,#74521,#74522,#74523,#74524,#74525,
#74526,#74527,#74528,#74529,#74530,#74531,#74532,#74533,#74534,#74535,#74536,
#74537,#74538,#74539,#74540,#74541,#74542,#74543,#74544,#74545,#74546,#74547,
#74548,#74549,#74550,#74551,#74552,#74553,#74554,#74555,#74556,#74557,#74558,
#74559,#74560,#74561,#74562,#74563,#74564,#74565,#74566,#74567,#74568,#74569,
#74570,#74571,#74572,#74573,#74574,#74575,#74576,#74577,#74578,#74579,#74580,
#74581,#74582,#74583,#74584,#74585,#74586,#74587,#74588,#74589,#74590,#74591,
#74592,#74593,#74594,#74595,#74596,#74597,#74598,#74599,#74600,#74601,#74602,
#74603,#74604,#74605,#74606,#74607,#74608,#74609,#74610,#74611,#74612,#74613,
#74614,#74615,#74616,#74617,#74618,#74619,#74620,#74621,#74622,#74623,#74624,
#74625,#74626,#74627),.UNSPECIFIED.,.F.,.F.,(4,2,2,2,2,2,2,2,2,2,2,2,2,
2,2,2,2,2,2,2,2,2,2,2,2,2,2,2,2,2,2,2,2,2,2,2,2,2,2,2,2,2,2,2,2,2,2,2,2,
2,2,2,2,2,2,2,2,2,2,2,2,2,2,2,2,2,2,2,2,2,2,2,2,2,2,2,2,2,2,2,2,2,2,2,2,
2,2,2,2,2,2,2,2,2,2,2,2,2,2,2,2,2,2,2,2,2,2,2,2,2,2,2,2,2,2,2,2,2,2,2,2,
2,2,2,4),(-2.66802149891279,-2.65996458342106,-2.65560732822634,-2.65419431785302,
-2.65312705204955,-2.65209682921456,-2.65091690148876,-2.64899166169616,
-2.64292604677928,-2.64164402158647,-2.63384352312468,-2.58064371327289,
-2.56289863577731,-2.55206075228039,-2.54875223902499,-2.54666532087034,
-2.54472890007616,-2.54221746690857,-2.53802604302116,-2.50852862303808,
-2.46741476353145,-2.45198071083895,-2.446566520425,-2.44396770674802,-2.4418610274011,
-2.44064831929846,-2.44064520469193,-2.44064207103828,-2.44063891828999,
-2.44063574642833,-2.4406325552362,-2.4406293446271,-2.44062611448397,-2.44062286459684,
-2.44061959475947,-2.44061630481875,-2.44061299472082,-2.44060966428502,
-2.44060632625828,-2.44060297370119,-2.44059959991487,-2.440596193339,-2.4395692317791,
-2.43819161733589,-2.43533418909548,-2.3992426131968,-2.36651413632511,
-2.34401631510754,-2.33837088445508,-2.33580095458918,-2.33386255053541,
-2.33203518178347,-2.32949118310903,-2.3228378179571,-2.26713559001317,
-2.24299761845435,-2.23215335381526,-2.2299079283935,-2.22865728322776,
-2.22758522498347,-2.22622936305462,-2.22408468155608,-2.21306506631437,
-2.16179724453626,-2.13310351536653,-2.12667124165372,-2.12396258478076,
-2.12200071722641,-2.12020780508928,-2.11734208474587,-2.11045420999899,
-2.0574066039162,-2.03147148976289,-2.02015654662414,-2.01788340882972,
-2.01662675056411,-2.01555527890836,-2.01420747533148,-2.01158600802693,
-1.99554933897305,-1.99020921886958,-1.97566181123813,-1.94276577714998,
-1.92619714808673,-1.91588354880024,-1.91263416695763,-1.91056044864088,
-1.90861942221413,-1.90607782968398,-1.90178219760266,-1.86666137899937,
-1.81773799092039,-1.80798026585771,-1.80580471181151,-1.80456933329518,
-1.80349536195426,-1.80211751978968,-1.79925935418478,-1.76331272716668,
-1.73052944568667,-1.70794918515225,-1.70229232727367,-1.69972013924318,
-1.6977812296767,-1.6959542644931,-1.69341224028618,-1.68677247458836,-1.63092250795175,
-1.59808291707098,-1.59453631026601,-1.59303192828603,-1.59194040903838,
-1.59091292144257,-1.58916250110634,-1.58438291672268,-1.5472057861471,
-1.49693562938493,-1.49053314054903,-1.48782935163067,-1.4858682149485,
-1.48407404461922,-1.48120211525056,-1.47427756954005,-1.42170690742326,
-1.40858075324139),.UNSPECIFIED.);
#790=B_SPLINE_CURVE_WITH_KNOTS('',3,(#74629,#74630,#74631,#74632,#74633,
#74634,#74635,#74636,#74637,#74638),.UNSPECIFIED.,.F.,.F.,(4,1,1,1,1,1,
1,4),(-60.0402340406592,-59.9301869977125,-58.9313505477506,-57.9325140977887,
-56.9336776478269,-55.934841197865,-54.9360047479031,-54.1065275198801),
 .UNSPECIFIED.);
#791=B_SPLINE_CURVE_WITH_KNOTS('',3,(#74639,#74640,#74641,#74642,#74643,
#74644,#74645,#74646,#74647,#74648,#74649,#74650,#74651,#74652,#74653,#74654,
#74655,#74656,#74657,#74658,#74659,#74660),.UNSPECIFIED.,.F.,.F.,(4,2,2,
2,2,2,2,2,2,2,4),(-2.66747056838221,-2.64324040236149,-2.63610839841556,
-2.63431747142202,-2.63310249420984,-2.63209340562307,-2.6310188153633,
-2.62963276479483,-2.62673172851018,-2.59981102814518,-2.59336897902399),
 .UNSPECIFIED.);
#792=B_SPLINE_CURVE_WITH_KNOTS('',3,(#74665,#74666,#74667,#74668,#74669,
#74670,#74671,#74672,#74673,#74674,#74675,#74676,#74677,#74678,#74679,#74680,
#74681,#74682,#74683,#74684,#74685,#74686,#74687,#74688,#74689,#74690,#74691,
#74692,#74693,#74694,#74695,#74696,#74697,#74698,#74699,#74700,#74701,#74702,
#74703,#74704,#74705,#74706,#74707,#74708,#74709,#74710,#74711,#74712,#74713,
#74714,#74715,#74716,#74717,#74718,#74719,#74720,#74721,#74722,#74723,#74724,
#74725,#74726,#74727,#74728,#74729,#74730,#74731,#74732,#74733,#74734,#74735,
#74736,#74737,#74738,#74739,#74740,#74741,#74742,#74743,#74744,#74745,#74746,
#74747,#74748,#74749,#74750,#74751,#74752,#74753,#74754,#74755,#74756,#74757,
#74758,#74759,#74760,#74761,#74762,#74763,#74764,#74765,#74766,#74767,#74768,
#74769,#74770,#74771,#74772,#74773,#74774,#74775,#74776,#74777,#74778,#74779,
#74780,#74781,#74782,#74783,#74784,#74785,#74786,#74787,#74788,#74789,#74790,
#74791,#74792,#74793,#74794,#74795,#74796,#74797,#74798,#74799,#74800,#74801,
#74802,#74803,#74804,#74805,#74806,#74807,#74808,#74809,#74810,#74811,#74812,
#74813,#74814,#74815,#74816,#74817,#74818,#74819,#74820,#74821,#74822,#74823,
#74824,#74825,#74826,#74827,#74828,#74829,#74830,#74831,#74832,#74833,#74834,
#74835,#74836,#74837,#74838,#74839,#74840,#74841,#74842,#74843,#74844,#74845,
#74846,#74847,#74848,#74849,#74850,#74851,#74852,#74853,#74854,#74855,#74856,
#74857,#74858,#74859,#74860,#74861,#74862,#74863,#74864,#74865,#74866,#74867,
#74868,#74869,#74870,#74871,#74872,#74873,#74874,#74875,#74876,#74877,#74878,
#74879,#74880,#74881,#74882,#74883,#74884,#74885,#74886,#74887,#74888,#74889,
#74890,#74891,#74892,#74893,#74894,#74895,#74896,#74897,#74898,#74899,#74900,
#74901,#74902,#74903,#74904),.UNSPECIFIED.,.F.,.F.,(4,2,2,2,2,2,2,2,2,2,
2,2,2,2,2,2,2,2,2,2,2,2,2,2,2,2,2,2,2,2,2,2,2,2,2,2,2,2,2,2,2,2,2,2,2,2,
2,2,2,2,2,2,2,2,2,2,2,2,2,2,2,2,2,2,2,2,2,2,2,2,2,2,2,2,2,2,2,2,2,2,2,2,
2,2,2,2,2,2,2,2,2,2,2,2,2,2,2,2,2,2,2,2,2,2,2,2,2,2,2,2,2,2,2,2,2,2,2,2,
2,4),(-1.40843520122759,-1.38234929436498,-1.36900905915055,-1.3654540019979,
-1.36331283927105,-1.36139154949988,-1.35894820923574,-1.35507363855925,
-1.33399939059767,-1.27618325037938,-1.261222380279,-1.25887432383507,-1.2574725015804,
-1.25639309875386,-1.2551864172719,-1.25314025936278,-1.24508269079824,
-1.22990316159912,-1.19000605476775,-1.15896149866968,-1.15473986411574,
-1.15221987285824,-1.15028241698707,-1.14819985476394,-1.14490988401863,
-1.13423600901413,-1.11686427510417,-1.06815962875071,-1.0616448088961,
-1.04902152617613,-1.04678573062594,-1.04540227320803,-1.04432782403015,
-1.04309628690015,-1.04093790540806,-1.03142591956689,-0.982271267862854,
-0.947074884913862,-0.942778461482244,-0.940236797658543,-0.938295934407803,
-0.936222600497801,-0.932974258368066,-0.922667560803234,-0.906115749914522,
-0.87326380443128,-0.860347435873508,-0.837642264741501,-0.834788611155627,
-0.833411808582419,-0.832338110264254,-0.831102447418038,-0.828924947134709,
-0.819134910169642,-0.770223736401356,-0.735105941467411,-0.730810954169608,
-0.728269844415247,-0.72632923408081,-0.724256005350361,-0.721007483512324,
-0.71069731215435,-0.69413716132622,-0.661280329478122,-0.647507728962088,
-0.640735546171248,-0.638905965280025,-0.625192231067182,-0.622901959248708,
-0.621517252313713,-0.620440276297059,-0.619224220890304,-0.617135131191565,
-0.608547985552004,-0.591852209341912,-0.549940166263519,-0.522879829308167,
-0.518757257096096,-0.516266556573872,-0.514333942997878,-0.512238984866759,
-0.508891489621154,-0.497683856649682,-0.479085549244681,-0.436433318725784,
-0.41374922225421,-0.410899941218018,-0.409524105866194,-0.40845062388991,
-0.407214602033347,-0.40503501200496,-0.395211333805982,-0.346336012184542,
-0.311232573450771,-0.306938283389392,-0.304397547223245,-0.302457199773498,
-0.300384230154729,-0.297136068926355,-0.286826659398029,-0.270267368247141,
-0.237928974445208,-0.201815752245152,-0.198960572232045,-0.197583654521324,
-0.196557124730904,-0.195363751317161,-0.19338085248251,-0.190941175898945,
-0.185983016961778,-0.172433086751189,-0.149616938249916,-0.103071425770781,
-0.0958751453617127,-0.0929586840934602,-0.0911568835027484,-0.0892033560504339,
-0.0865388181216794,-0.0803613062889754,-0.0750411156564984),
 .UNSPECIFIED.);
#793=B_SPLINE_CURVE_WITH_KNOTS('',3,(#74905,#74906,#74907,#74908,#74909,
#74910,#74911,#74912,#74913,#74914,#74915,#74916,#74917,#74918,#74919,#74920,
#74921,#74922,#74923,#74924,#74925,#74926,#74927,#74928,#74929,#74930,#74931,
#74932,#74933,#74934,#74935,#74936,#74937,#74938,#74939,#74940,#74941,#74942,
#74943,#74944,#74945,#74946,#74947,#74948,#74949,#74950,#74951,#74952,#74953,
#74954,#74955,#74956,#74957,#74958,#74959,#74960,#74961,#74962,#74963,#74964,
#74965,#74966,#74967,#74968,#74969,#74970,#74971,#74972,#74973,#74974,#74975,
#74976,#74977,#74978,#74979,#74980,#74981,#74982,#74983,#74984,#74985,#74986,
#74987,#74988,#74989,#74990,#74991,#74992,#74993,#74994,#74995,#74996,#74997,
#74998,#74999,#75000,#75001,#75002,#75003,#75004,#75005,#75006,#75007,#75008,
#75009,#75010,#75011,#75012,#75013,#75014,#75015,#75016,#75017,#75018,#75019,
#75020,#75021,#75022,#75023,#75024,#75025,#75026,#75027,#75028,#75029,#75030,
#75031,#75032,#75033,#75034,#75035,#75036,#75037,#75038,#75039,#75040,#75041,
#75042,#75043,#75044,#75045,#75046,#75047,#75048,#75049,#75050,#75051,#75052,
#75053,#75054,#75055,#75056,#75057,#75058,#75059,#75060,#75061,#75062,#75063,
#75064,#75065,#75066,#75067,#75068,#75069,#75070,#75071,#75072,#75073,#75074,
#75075,#75076,#75077,#75078,#75079,#75080,#75081,#75082,#75083,#75084,#75085,
#75086,#75087,#75088,#75089,#75090,#75091,#75092,#75093,#75094,#75095,#75096,
#75097,#75098,#75099,#75100,#75101,#75102,#75103,#75104,#75105,#75106,#75107,
#75108,#75109,#75110,#75111,#75112,#75113,#75114,#75115,#75116,#75117,#75118,
#75119,#75120,#75121,#75122,#75123,#75124,#75125,#75126,#75127,#75128,#75129,
#75130,#75131,#75132,#75133,#75134),.UNSPECIFIED.,.F.,.F.,(4,2,2,2,2,2,
2,2,2,2,2,2,2,2,2,2,2,2,2,2,2,2,2,2,2,2,2,2,2,2,2,2,2,2,2,2,2,2,2,2,2,2,
2,2,2,2,2,2,2,2,2,2,2,2,2,2,2,2,2,2,2,2,2,2,2,2,2,2,2,2,2,2,2,2,2,2,2,2,
2,2,2,2,2,2,2,2,2,2,2,2,2,2,2,2,2,2,2,2,2,2,2,2,2,2,2,2,2,2,2,2,2,2,2,2,
4),(-2.59336897902399,-2.58612775773752,-2.57460692284161,-2.54603037275735,
-2.53213217693245,-2.52852862917153,-2.52637674652784,-2.52445745754336,
-2.5220324026772,-2.5173006069789,-2.47986237414341,-2.42951076665685,-2.42303686747642,
-2.42114543005634,-2.42013445334268,-2.419061171705,-2.41768947020732,-2.41549247588205,
-2.40365533751416,-2.34625797232683,-2.32969428769209,-2.31938348363044,
-2.31613483212643,-2.31406154378695,-2.31212089445579,-2.30957975909593,
-2.3052848176617,-2.27015873082236,-2.22120715913026,-2.21149608652536,
-2.20932403380151,-2.20808957524292,-2.20701571868636,-2.20563712748466,
-2.20277431791584,-2.1671499722037,-2.13426642530221,-2.1177090732739,-2.10740103365598,
-2.10415262657573,-2.10207934365023,-2.10013859360948,-2.09759717375137,
-2.09330140936512,-2.05812248547131,-2.0090030328744,-1.99948550962677,
-1.99732688032396,-1.99609534933601,-1.99502100607967,-1.99363780696882,
-1.99140265782503,-1.97878987261475,-1.97427160519009,-1.92390177362098,
-1.90628135760737,-1.89549917621213,-1.89219745169104,-1.89011245776445,
-1.88817619708699,-1.88566266851789,-1.88146268977052,-1.85136029210321,
-1.79974352603178,-1.78774374617407,-1.785432846755,-1.78416808589976,-1.78309734572312,
-1.78176010813924,-1.77967596377317,-1.76959020978519,-1.76409154505887,
-1.75666401725485,-1.74315683683923,-1.71027514660382,-1.69372148045322,
-1.68341493028853,-1.68016656398209,-1.67809320405943,-1.67615230956651,
-1.67361059610496,-1.66931410131359,-1.63409706808228,-1.58485217209879,
-1.57547452778713,-1.5733257394765,-1.5720963294015,-1.57102156821656,-1.56963484364631,
-1.56738812898032,-1.55455522106751,-1.55238921011321,-1.50510882210855,
-1.47658468319908,-1.47017272022229,-1.46746753569891,-1.46550633507785,
-1.46371275966823,-1.46084320709142,-1.45393175833352,-1.40120067523501,
-1.37504634358037,-1.36367583392588,-1.36139955533112,-1.36014223469209,
-1.35907084944986,-1.35772398303932,-1.35510677225267,-1.33914478487925,
-1.3342007853959,-1.32855480469969,-1.28159544034006,-1.28015025094885,
-1.26111046282178,-1.25973256582632),.UNSPECIFIED.);
#794=B_SPLINE_CURVE_WITH_KNOTS('',3,(#75140,#75141,#75142,#75143,#75144,
#75145,#75146,#75147,#75148,#75149,#75150,#75151,#75152,#75153,#75154,#75155),
 .UNSPECIFIED.,.F.,.F.,(4,2,2,2,2,2,2,4),(-0.0747818727151328,-0.0742459240434196,
-0.0731681029222417,-0.0719558860471734,-0.0698841331767219,-0.0615139050350039,
-0.0454480673956834,-0.000629549970892275),.UNSPECIFIED.);
#795=B_SPLINE_CURVE_WITH_KNOTS('',3,(#75156,#75157,#75158,#75159,#75160,
#75161,#75162,#75163,#75164,#75165,#75166,#75167,#75168,#75169,#75170,#75171,
#75172,#75173,#75174,#75175,#75176,#75177,#75178,#75179,#75180,#75181,#75182,
#75183,#75184,#75185,#75186,#75187,#75188,#75189,#75190,#75191,#75192,#75193,
#75194,#75195,#75196,#75197,#75198,#75199,#75200,#75201,#75202,#75203,#75204,
#75205,#75206,#75207,#75208,#75209,#75210,#75211,#75212,#75213,#75214,#75215,
#75216,#75217,#75218,#75219,#75220,#75221,#75222,#75223,#75224,#75225,#75226,
#75227,#75228,#75229,#75230,#75231,#75232,#75233,#75234,#75235,#75236,#75237,
#75238,#75239,#75240,#75241,#75242,#75243,#75244,#75245,#75246,#75247,#75248,
#75249,#75250,#75251,#75252,#75253,#75254,#75255,#75256,#75257,#75258,#75259,
#75260,#75261,#75262,#75263,#75264,#75265,#75266,#75267,#75268,#75269,#75270,
#75271,#75272,#75273,#75274,#75275,#75276,#75277,#75278,#75279,#75280,#75281,
#75282,#75283,#75284,#75285,#75286,#75287,#75288,#75289,#75290,#75291,#75292,
#75293,#75294,#75295,#75296,#75297,#75298,#75299,#75300,#75301,#75302,#75303,
#75304,#75305,#75306,#75307,#75308,#75309,#75310,#75311,#75312,#75313,#75314,
#75315,#75316,#75317,#75318,#75319,#75320,#75321,#75322,#75323,#75324,#75325,
#75326,#75327,#75328,#75329,#75330,#75331,#75332,#75333,#75334,#75335,#75336,
#75337,#75338,#75339,#75340,#75341,#75342,#75343,#75344,#75345,#75346,#75347,
#75348,#75349,#75350,#75351,#75352,#75353,#75354,#75355,#75356,#75357,#75358,
#75359,#75360,#75361,#75362,#75363,#75364,#75365,#75366,#75367,#75368,#75369,
#75370,#75371,#75372,#75373,#75374,#75375,#75376,#75377,#75378,#75379),
 .UNSPECIFIED.,.F.,.F.,(4,2,2,2,2,2,2,2,2,2,2,2,2,2,2,2,2,2,2,2,2,2,2,2,
2,2,2,2,2,2,2,2,2,2,2,2,2,2,2,2,2,2,2,2,2,2,2,2,2,2,2,2,2,2,2,2,2,2,2,2,
2,2,2,2,2,2,2,2,2,2,2,2,2,2,2,2,2,2,2,2,2,2,2,2,2,2,2,2,2,2,2,2,2,2,2,2,
2,2,2,2,2,2,2,2,2,2,2,2,2,2,2,4),(-2.66773930540004,-2.64241116651683,-2.63928395192308,
-2.63713771430998,-2.63533677411038,-2.63342268369052,-2.63105334550721,
-2.62741952032345,-2.61031288541215,-2.59812141782425,-2.56892054787406,
-2.53462366403773,-2.53107188279988,-2.52956695134289,-2.52847565367427,
-2.52744886994475,-2.52570071393307,-2.52093343051611,-2.48338424598238,
-2.45585429059528,-2.43890003757105,-2.4319395124763,-2.42667070342962,
-2.42418246266504,-2.42234810064803,-2.42053096910391,-2.41802500843694,
-2.41160546890512,-2.35378688144598,-2.33102452161715,-2.32055935487983,
-2.31833768920478,-2.31709239399665,-2.31602001809181,-2.31465743126096,
-2.31249017417579,-2.30109422186171,-2.25006719077044,-2.22154459090812,
-2.21513337203888,-2.21242861569957,-2.21046776707741,-2.20867454222068,
-2.20580561291208,-2.19889598835342,-2.14617228536373,-2.12002416897991,
-2.1086561187757,-2.10638028414092,-2.10512320225078,-2.10405201652662,
-2.10270539594568,-2.1000886481999,-2.08412916043406,-2.07850644238329,
-2.06415895635759,-2.03127212101885,-2.01470967563004,-2.00439947158316,
-2.00115091795063,-1.99907767016636,-1.99713704340873,-1.9945959154069,
-1.99030093665389,-1.95516790019283,-1.90619370162443,-1.89651019123151,
-1.89434005987186,-1.89310603453091,-1.89203213189743,-1.89065292780709,
-1.88843091391134,-1.87606365563223,-1.87297920045015,-1.87277976154329,
-1.86591263585554,-1.85218003620042,-1.81929740647948,-1.80274167262832,
-1.79243430196009,-1.78918592555969,-1.78711261892362,-1.78517181627456,
-1.78263028364007,-1.77833423025561,-1.74313950070793,-1.69396848415567,
-1.68450892814661,-1.68235436241328,-1.68112370972071,-1.68004920009232,
-1.6786645603133,-1.67577105398807,-1.64973656568661,-1.61156942222171,
-1.58254141965607,-1.57814579748564,-1.57582221950715,-1.57391060877851,
-1.57168647965745,-1.56785821382003,-1.55279682990344,-1.50062826088653,
-1.48178263607802,-1.4724867746221,-1.47034387109809,-1.46911575820303,
-1.46804078187306,-1.46665199933797,-1.46373737361904,-1.43369111484034,
-1.40843520122759),.UNSPECIFIED.);
#796=B_SPLINE_CURVE_WITH_KNOTS('',3,(#75381,#75382,#75383,#75384,#75385,
#75386,#75387,#75388,#75389,#75390,#75391,#75392,#75393,#75394,#75395,#75396,
#75397,#75398,#75399,#75400,#75401,#75402,#75403,#75404,#75405,#75406,#75407,
#75408,#75409,#75410,#75411,#75412,#75413,#75414,#75415,#75416,#75417,#75418,
#75419,#75420,#75421,#75422,#75423,#75424,#75425,#75426,#75427,#75428,#75429,
#75430,#75431,#75432,#75433,#75434,#75435,#75436,#75437,#75438,#75439,#75440,
#75441,#75442,#75443,#75444,#75445,#75446,#75447,#75448,#75449,#75450,#75451,
#75452,#75453,#75454,#75455,#75456,#75457,#75458,#75459,#75460,#75461,#75462,
#75463,#75464,#75465,#75466,#75467,#75468,#75469,#75470,#75471,#75472,#75473,
#75474,#75475,#75476,#75477,#75478,#75479,#75480,#75481,#75482,#75483,#75484,
#75485,#75486,#75487,#75488,#75489,#75490,#75491,#75492,#75493,#75494,#75495,
#75496,#75497,#75498,#75499,#75500,#75501,#75502,#75503,#75504,#75505,#75506,
#75507,#75508,#75509,#75510,#75511,#75512,#75513,#75514,#75515,#75516,#75517,
#75518,#75519,#75520,#75521,#75522,#75523,#75524,#75525,#75526,#75527,#75528,
#75529,#75530,#75531,#75532,#75533,#75534,#75535,#75536,#75537,#75538,#75539,
#75540,#75541,#75542,#75543,#75544,#75545,#75546,#75547,#75548,#75549,#75550,
#75551,#75552,#75553,#75554,#75555,#75556,#75557,#75558,#75559,#75560,#75561,
#75562,#75563,#75564,#75565,#75566,#75567,#75568,#75569,#75570,#75571,#75572,
#75573,#75574,#75575,#75576,#75577,#75578,#75579,#75580,#75581,#75582,#75583,
#75584,#75585,#75586,#75587,#75588,#75589,#75590,#75591,#75592,#75593,#75594,
#75595,#75596,#75597,#75598),.UNSPECIFIED.,.F.,.F.,(4,2,2,2,2,2,2,2,2,2,
2,2,2,2,2,2,2,2,2,2,2,2,2,2,2,2,2,2,2,2,2,2,2,2,2,2,2,2,2,2,2,2,2,2,2,2,
2,2,2,2,2,2,2,2,2,2,2,2,2,2,2,2,2,2,2,2,2,2,2,2,2,2,2,2,2,2,2,2,2,2,2,2,
2,2,2,2,2,2,2,2,2,2,2,2,2,2,2,2,2,2,2,2,2,2,2,2,2,2,4),(-1.25973256582632,
-1.25734927536444,-1.25494051512531,-1.25302276260143,-1.25086057234657,
-1.24721078439067,-1.23275868433367,-1.18237142310263,-1.15270373796546,
-1.14978925033321,-1.14840048727113,-1.14732550086462,-1.14609735761107,
-1.14395434257905,-1.13465739666924,-1.11580594357347,-1.07535275874928,
-1.0630740852536,-1.04849430481256,-1.04470833580197,-1.04249388523533,
-1.04058159978212,-1.03824591976207,-1.03379285064424,-1.00275690956424,
-0.954779868459052,-0.940190390243041,-0.937858015806157,-0.936460774833188,
-0.935381980597219,-0.934172725913621,-0.932115032158586,-0.923919821841095,
-0.908354200208845,-0.866772480596383,-0.854678395852469,-0.836943442398868,
-0.833268238942155,-0.830885873611517,-0.828970408497621,-0.826790607377273,
-0.823061326865718,-0.807597276748613,-0.755884060562644,-0.728679220408929,
-0.725775768173161,-0.724389116142881,-0.723314311240784,-0.722084748327888,
-0.719935436921174,-0.710551821461474,-0.661283547357181,-0.626053184033462,
-0.62175620112068,-0.61921433348283,-0.617273387810849,-0.615200036826116,
-0.611951816094066,-0.601646751784312,-0.585098750021702,-0.552249351195666,
-0.539730922023649,-0.51662183427344,-0.51376440127891,-0.512386830460004,
-0.511313028808089,-0.510077806743987,-0.507902421998602,-0.498144051760086,
-0.44920433462688,-0.414077902096759,-0.409781931034492,-0.407240494728494,
-0.405299782127785,-0.403226586768878,-0.399978414986767,-0.389671864211867,
-0.373119914740638,-0.340269276295497,-0.327232030559009,-0.318524919112912,
-0.30421425517336,-0.301893582119799,-0.300499910548861,-0.2994217613812,
-0.298210870599363,-0.296145157880832,-0.287849400271933,-0.271996907622163,
-0.225995378602473,-0.20164681590449,-0.197627685049602,-0.195167512852649,
-0.193296806704232,-0.191269131835227,-0.188079691277217,-0.18432709544764,
-0.177197803230122,-0.159650714105301,-0.109620595682326,-0.0924449856537553,
-0.0897803292526254,-0.0884234221347708,-0.0873515073188859,-0.0861021507250372,
-0.0838618226893698,-0.0730958619668398,-0.0492411657667594,-0.000629479043906068),
 .UNSPECIFIED.);
#797=B_SPLINE_CURVE_WITH_KNOTS('',3,(#75599,#75600,#75601,#75602,#75603,
#75604,#75605,#75606,#75607,#75608,#75609,#75610,#75611,#75612,#75613,#75614,
#75615,#75616,#75617,#75618,#75619,#75620),.UNSPECIFIED.,.F.,.F.,(4,2,2,
2,2,2,2,2,2,2,4),(-2.66782448542482,-2.66003056299692,-2.65473405888332,
-2.65229065144145,-2.65040877439129,-2.64856804455869,-2.6467416187617,
-2.644201195173,-2.63900996170188,-2.62649959238965,-2.59341035609829),
 .UNSPECIFIED.);
#798=B_SPLINE_CURVE_WITH_KNOTS('',3,(#75625,#75626,#75627,#75628,#75629,
#75630,#75631,#75632,#75633,#75634,#75635,#75636,#75637,#75638,#75639,#75640,
#75641,#75642,#75643,#75644,#75645,#75646,#75647,#75648,#75649,#75650,#75651,
#75652,#75653,#75654,#75655,#75656,#75657,#75658,#75659,#75660,#75661,#75662,
#75663,#75664,#75665,#75666,#75667,#75668,#75669,#75670,#75671,#75672,#75673,
#75674,#75675,#75676,#75677,#75678,#75679,#75680,#75681,#75682,#75683,#75684,
#75685,#75686,#75687,#75688,#75689,#75690,#75691,#75692,#75693,#75694,#75695,
#75696,#75697,#75698,#75699,#75700,#75701,#75702,#75703,#75704,#75705,#75706,
#75707,#75708,#75709,#75710,#75711,#75712,#75713,#75714,#75715,#75716,#75717,
#75718,#75719,#75720,#75721,#75722,#75723,#75724,#75725,#75726,#75727,#75728,
#75729,#75730,#75731,#75732,#75733,#75734,#75735,#75736,#75737,#75738,#75739,
#75740,#75741,#75742,#75743,#75744,#75745,#75746,#75747,#75748,#75749,#75750,
#75751,#75752,#75753,#75754,#75755,#75756,#75757,#75758,#75759,#75760,#75761,
#75762,#75763,#75764,#75765,#75766,#75767,#75768,#75769,#75770,#75771,#75772,
#75773,#75774,#75775,#75776,#75777,#75778,#75779,#75780,#75781,#75782,#75783,
#75784,#75785,#75786,#75787,#75788,#75789,#75790,#75791,#75792,#75793,#75794,
#75795,#75796,#75797,#75798,#75799,#75800,#75801,#75802,#75803,#75804,#75805,
#75806,#75807,#75808,#75809,#75810,#75811,#75812,#75813,#75814,#75815,#75816,
#75817,#75818,#75819,#75820,#75821,#75822,#75823,#75824,#75825,#75826,#75827,
#75828,#75829,#75830,#75831,#75832,#75833,#75834,#75835,#75836,#75837,#75838,
#75839,#75840,#75841,#75842,#75843,#75844,#75845,#75846,#75847,#75848,#75849,
#75850),.UNSPECIFIED.,.F.,.F.,(4,2,2,2,2,2,2,2,2,2,2,2,2,2,2,2,2,2,2,2,
2,2,2,2,2,2,2,2,2,2,2,2,2,2,2,2,2,2,2,2,2,2,2,2,2,2,2,2,2,2,2,2,2,2,2,2,
2,2,2,2,2,2,2,2,2,2,2,2,2,2,2,2,2,2,2,2,2,2,2,2,2,2,2,2,2,2,2,2,2,2,2,2,
2,2,2,2,2,2,2,2,2,2,2,2,2,2,2,2,2,2,2,2,4),(-1.40853711338947,-1.36768270255549,
-1.35578956926343,-1.35125426050673,-1.3479456909352,-1.34648313700913,
-1.34539838134693,-1.34420943539953,-1.34224339368389,-1.33583797627915,
-1.33428199270909,-1.31969474787633,-1.26065036180123,-1.24633998830998,
-1.2425781217769,-1.24036918321174,-1.23845643661397,-1.2361135976534,-1.23162645537363,
-1.19926315773716,-1.15907925242498,-1.15414634840198,-1.13819555014462,
-1.13557886251389,-1.13423207991095,-1.13316066320953,-1.13190319752587,
-1.12962637058364,-1.11824778254315,-1.09205969086143,-1.03933108993612,
-1.03241647585102,-1.02954634069093,-1.02775261667785,-1.02579143240917,
-1.02308659010719,-1.01667693114487,-0.988176704974518,-0.937243776280263,
-0.925759998176468,-0.923587350311914,-0.922222991473029,-0.921150292215095,
-0.919905852199562,-0.917688723844539,-0.907300008974863,-0.884808705648799,
-0.8264863374873,-0.820127956641291,-0.817631925077921,-0.815817166197529,
-0.813871711075465,-0.811257075627084,-0.805364991996072,-0.781011902670562,
-0.730339777255363,-0.714121237846193,-0.711492998487255,-0.71014378163785,
-0.709072270871095,-0.707816827755718,-0.705549074063951,-0.694326253900503,
-0.668747008170932,-0.615147894274237,-0.608301667084345,-0.60544289883552,
-0.603651322368631,-0.601688493056375,-0.598974045732415,-0.592506768400468,
-0.538333992281918,-0.502384842989942,-0.499521337710469,-0.498142551109291,
-0.497068604359849,-0.495834120598664,-0.493662197067835,-0.483954892154799,
-0.434970205919605,-0.399813904055265,-0.39552587454896,-0.392986701772883,
-0.391046314133845,-0.388972103828962,-0.385719494932899,-0.375374808873267,
-0.358738674649535,-0.325817684217832,-0.30777021760443,-0.290180233967672,
-0.287500587862765,-0.286140445965236,-0.285068237708011,-0.283821132051401,
-0.281591270946103,-0.270996363690899,-0.247766310106086,-0.192021882931062,
-0.184529990832604,-0.181562890210456,-0.179751487614206,-0.177920924583202,
-0.175416652164948,-0.17009691241572,-0.163034149925774,-0.145722466034039,
-0.0976541025404786,-0.0933269148221475,-0.0921194914598723,-0.0779498329751376,
-0.0756372155382893,-0.0747818727151328),.UNSPECIFIED.);
#799=B_SPLINE_CURVE_WITH_KNOTS('',3,(#75851,#75852,#75853,#75854,#75855,
#75856,#75857,#75858,#75859,#75860,#75861,#75862,#75863,#75864,#75865,#75866,
#75867,#75868,#75869,#75870,#75871,#75872,#75873,#75874,#75875,#75876,#75877,
#75878,#75879,#75880,#75881,#75882,#75883,#75884,#75885,#75886,#75887,#75888,
#75889,#75890,#75891,#75892,#75893,#75894,#75895,#75896,#75897,#75898,#75899,
#75900,#75901,#75902,#75903,#75904,#75905,#75906,#75907,#75908,#75909,#75910,
#75911,#75912,#75913,#75914,#75915,#75916,#75917,#75918,#75919,#75920,#75921,
#75922,#75923,#75924,#75925,#75926,#75927,#75928,#75929,#75930,#75931,#75932,
#75933,#75934,#75935,#75936,#75937,#75938,#75939,#75940,#75941,#75942,#75943,
#75944,#75945,#75946,#75947,#75948,#75949,#75950,#75951,#75952,#75953,#75954,
#75955,#75956,#75957,#75958,#75959,#75960,#75961,#75962,#75963,#75964,#75965,
#75966,#75967,#75968,#75969,#75970,#75971,#75972,#75973,#75974,#75975,#75976,
#75977,#75978,#75979,#75980,#75981,#75982,#75983,#75984,#75985,#75986,#75987,
#75988,#75989,#75990,#75991,#75992,#75993,#75994,#75995,#75996,#75997,#75998,
#75999,#76000,#76001,#76002,#76003,#76004,#76005,#76006,#76007,#76008,#76009,
#76010,#76011,#76012,#76013,#76014,#76015,#76016,#76017,#76018,#76019,#76020,
#76021,#76022,#76023,#76024,#76025,#76026,#76027,#76028,#76029,#76030,#76031,
#76032,#76033,#76034,#76035,#76036,#76037,#76038,#76039,#76040,#76041,#76042,
#76043,#76044,#76045,#76046,#76047,#76048,#76049,#76050,#76051,#76052,#76053,
#76054,#76055,#76056,#76057,#76058,#76059,#76060,#76061,#76062,#76063,#76064,
#76065,#76066,#76067,#76068,#76069,#76070,#76071,#76072,#76073,#76074,#76075,
#76076,#76077,#76078,#76079,#76080,#76081,#76082,#76083,#76084,#76085,#76086,
#76087,#76088,#76089,#76090,#76091,#76092,#76093,#76094,#76095,#76096,#76097,
#76098,#76099,#76100,#76101,#76102,#76103,#76104,#76105,#76106,#76107,#76108,
#76109,#76110,#76111,#76112,#76113,#76114,#76115,#76116,#76117,#76118,#76119,
#76120),.UNSPECIFIED.,.F.,.F.,(4,2,2,2,2,2,2,2,2,2,2,2,2,2,2,2,2,2,2,2,
2,2,2,2,2,2,2,2,2,2,2,2,2,2,2,2,2,2,2,2,2,2,2,2,2,2,2,2,2,2,2,2,2,2,2,2,
2,2,2,2,2,2,2,2,2,2,2,2,2,2,2,2,2,2,2,2,2,2,2,2,2,2,2,2,2,2,2,2,2,2,2,2,
2,2,2,2,2,2,2,2,2,2,2,2,2,2,2,2,2,2,2,2,2,2,2,2,2,2,2,2,2,2,2,2,2,2,2,2,
2,2,2,2,2,2,4),(-2.59341035609829,-2.57482973281229,-2.55598714875694,-2.54669214216968,
-2.54454925113748,-2.54332111565175,-2.54224610013818,-2.54085724135978,
-2.53794236515546,-2.50824565034493,-2.45779622037755,-2.44830716136627,
-2.44369986741691,-2.43992075424202,-2.43775004254392,-2.43773434805528,
-2.43771810100957,-2.43770128128463,-2.43768386804235,-2.4376658396592,
-2.43764717373721,-2.43762784707113,-2.43760783566919,-2.43758711458412,
-2.43756565797438,-2.43754343913426,-2.43752042968978,-2.43750039340549,
-2.43747704310926,-2.43744983674674,-2.43741814627615,-2.43738124537686,
-2.4373382957925,-2.43728408358569,-2.43534335946234,-2.43280134459612,
-2.42850316409415,-2.39338170488472,-2.34442283443053,-2.33472342946418,
-2.33255224903429,-2.33131801687544,-2.33024418441593,-2.32886539790547,
-2.32600140177476,-2.29004808887267,-2.25728170633324,-2.23472083343327,
-2.22906723249113,-2.22649601649929,-2.22455763260498,-2.22273101060838,
-2.22018921976626,-2.21354860988395,-2.15774103602243,-2.13368050345915,
-2.12285772072217,-2.12061382038051,-2.11936361505868,-2.11829168136597,
-2.11693565306005,-2.1147901015043,-2.10375313026405,-2.05253679571314,
-2.02382742289741,-2.01739370999166,-2.0146850384666,-2.01272337486551,
-2.01093079668361,-2.00806593103643,-2.00118177306371,-1.94810593027268,
-1.92219927649779,-1.91089225080458,-1.90861979607212,-1.90736339337595,
-1.90629206552154,-1.90494434847348,-1.90232277186784,-1.8862807194765,
-1.88099085656435,-1.86640570341081,-1.83351383751184,-1.81694698925262,
-1.80663459172248,-1.80338563809073,-1.8013122049657,-1.79937145384903,
-1.79683023388239,-1.79253525853405,-1.75742339526241,-1.70851920848977,
-1.6987482631656,-1.6965720165787,-1.69533659221617,-1.69426280339793,-1.69288548608946,
-1.69002940945599,-1.66723137756675,-1.61162104754378,-1.5956093759142,
-1.59183989743885,-1.58965142381957,-1.58773722178025,-1.58536794699408,
-1.58173459654937,-1.56463773712466,-1.55656865460642,-1.52175804244607,
-1.4977085530994,-1.48688900275794,-1.48464539097727,-1.48339529293298,
-1.4823234182358,-1.48096742224301,-1.47830713863393,-1.46125353870752,
-1.44264161588998,-1.4096854119617,-1.39304017869419,-1.38269247931452,
-1.37943955830635,-1.37736530758679,-1.37542499394027,-1.37288608028755,
-1.36859888349708,-1.33401767631518,-1.27805192423931,-1.2737780967122,
-1.27210652013368,-1.27109449105814,-1.26999215497845,-1.26842723567567,
-1.26451471126435,-1.25986135129038),.UNSPECIFIED.);
#800=B_SPLINE_CURVE_WITH_KNOTS('',3,(#76126,#76127,#76128,#76129,#76130,
#76131,#76132,#76133,#76134,#76135,#76136,#76137,#76138,#76139,#76140,#76141,
#76142,#76143),.UNSPECIFIED.,.F.,.F.,(4,2,2,2,2,2,2,2,4),(-0.0751187349318719,
-0.0651106329348145,-0.0603739125176121,-0.0579481082617559,-0.0560290964025899,
-0.0538784373609023,-0.0516517499321186,-0.048329966890634,-0.00062898517661497),
 .UNSPECIFIED.);
#801=B_SPLINE_CURVE_WITH_KNOTS('',3,(#76144,#76145,#76146,#76147,#76148,
#76149,#76150,#76151,#76152,#76153,#76154,#76155,#76156,#76157,#76158,#76159,
#76160,#76161,#76162,#76163,#76164,#76165,#76166,#76167,#76168,#76169,#76170,
#76171,#76172,#76173,#76174,#76175,#76176,#76177,#76178,#76179,#76180,#76181,
#76182,#76183,#76184,#76185,#76186,#76187,#76188,#76189,#76190,#76191,#76192,
#76193,#76194,#76195,#76196,#76197,#76198,#76199,#76200,#76201,#76202,#76203,
#76204,#76205,#76206,#76207,#76208,#76209,#76210,#76211,#76212,#76213,#76214,
#76215,#76216,#76217,#76218,#76219,#76220,#76221,#76222,#76223,#76224,#76225,
#76226,#76227,#76228,#76229,#76230,#76231,#76232,#76233,#76234,#76235,#76236,
#76237,#76238,#76239,#76240,#76241,#76242,#76243,#76244,#76245,#76246,#76247,
#76248,#76249,#76250,#76251,#76252,#76253,#76254,#76255,#76256,#76257,#76258,
#76259,#76260,#76261,#76262,#76263,#76264,#76265,#76266,#76267,#76268,#76269,
#76270,#76271,#76272,#76273,#76274,#76275,#76276,#76277,#76278,#76279,#76280,
#76281,#76282,#76283,#76284,#76285,#76286,#76287,#76288,#76289,#76290,#76291,
#76292,#76293,#76294,#76295,#76296,#76297,#76298,#76299,#76300,#76301,#76302,
#76303,#76304,#76305,#76306,#76307,#76308,#76309,#76310,#76311,#76312,#76313,
#76314,#76315,#76316,#76317,#76318,#76319,#76320,#76321,#76322,#76323,#76324,
#76325,#76326,#76327,#76328,#76329,#76330,#76331,#76332,#76333,#76334,#76335,
#76336,#76337,#76338,#76339,#76340,#76341,#76342,#76343,#76344,#76345,#76346,
#76347,#76348,#76349,#76350,#76351,#76352,#76353,#76354,#76355,#76356,#76357,
#76358,#76359,#76360,#76361,#76362,#76363,#76364,#76365,#76366,#76367,#76368,
#76369),.UNSPECIFIED.,.F.,.F.,(4,2,2,2,2,2,2,2,2,2,2,2,2,2,2,2,2,2,2,2,
2,2,2,2,2,2,2,2,2,2,2,2,2,2,2,2,2,2,2,2,2,2,2,2,2,2,2,2,2,2,2,2,2,2,2,2,
2,2,2,2,2,2,2,2,2,2,2,2,2,2,2,2,2,2,2,2,2,2,2,2,2,2,2,2,2,2,2,2,2,2,2,2,
2,2,2,2,2,2,2,2,2,2,2,2,2,2,2,2,2,2,2,2,4),(-2.66780309434801,-2.62484505800817,
-2.6219108313024,-2.62022793742123,-2.61872288020446,-2.61763118378487,
-2.61660377922286,-2.61485403788078,-2.61007939121883,-2.57261984535515,
-2.55119597702224,-2.52285730101152,-2.51638402150457,-2.51425965737376,
-2.512179581606,-2.51024060531169,-2.50771316384361,-2.50346695702633,-2.47124361159917,
-2.43574887781677,-2.41831569260106,-2.40949761061823,-2.40739741601031,
-2.40616906546414,-2.40509386011329,-2.40370475397877,-2.4007893512284,
-2.3710053731005,-2.32035366152312,-2.30620902996869,-2.30265828682094,
-2.3004738999177,-2.29855864866291,-2.29618207295407,-2.29252624039311,
-2.27509632343502,-2.22285291979168,-2.20601392043731,-2.19737612072976,
-2.19528248952006,-2.19406512069525,-2.19298788184882,-2.19160398401279,
-2.18931741368778,-2.17569419079213,-2.17392046746541,-2.166804715018,-2.12338057659755,
-2.10479361976828,-2.09359066569597,-2.09024276176984,-2.08814715216989,
-2.08621366946873,-2.08372147533988,-2.07959565232913,-2.05244999275112,
-2.01051591878271,-1.99390430985192,-1.98534395402353,-1.98325643172913,
-1.98204042008085,-1.9809629033154,-1.97957674056477,-1.97728247970232,
-1.96350060092353,-1.95214312780525,-1.91150136399021,-1.89282467746958,
-1.88158325256089,-1.87823124900663,-1.87613472058105,-1.8742015077424,
-1.87171122179838,-1.86759192826074,-1.84070506459315,-1.79874615663962,
-1.78195714237243,-1.7733362968348,-1.77124398859113,-1.77002690865292,
-1.76894960247881,-1.76756520202095,-1.76527694171419,-1.7516191663709,
-1.7498803364374,-1.70251038386924,-1.67153423136465,-1.66708202205485,
-1.6647462893385,-1.66283370643507,-1.66061862546172,-1.65683088348565,
-1.64223557993222,-1.62996945749286,-1.58955643563185,-1.57070181848982,
-1.5614025671802,-1.55925918133821,-1.55803084022124,-1.55695569556991,
-1.55556673707924,-1.5526518886144,-1.52381225837565,-1.48570039543634,
-1.46817383401427,-1.45743214822732,-1.45413430823221,-1.45204979445138,
-1.45011261740564,-1.4475959658139,-1.44338651476126,-1.41291090387463,
-1.40853711338947),.UNSPECIFIED.);
#802=B_SPLINE_CURVE_WITH_KNOTS('',3,(#76371,#76372,#76373,#76374,#76375,
#76376,#76377,#76378,#76379,#76380,#76381,#76382,#76383,#76384,#76385,#76386,
#76387,#76388,#76389,#76390,#76391,#76392,#76393,#76394,#76395,#76396,#76397,
#76398,#76399,#76400,#76401,#76402,#76403,#76404,#76405,#76406,#76407,#76408,
#76409,#76410,#76411,#76412,#76413,#76414,#76415,#76416,#76417,#76418,#76419,
#76420,#76421,#76422,#76423,#76424,#76425,#76426,#76427,#76428,#76429,#76430,
#76431,#76432,#76433,#76434,#76435,#76436,#76437,#76438,#76439,#76440,#76441,
#76442,#76443,#76444,#76445,#76446,#76447,#76448,#76449,#76450,#76451,#76452,
#76453,#76454,#76455,#76456,#76457,#76458,#76459,#76460,#76461,#76462,#76463,
#76464,#76465,#76466,#76467,#76468,#76469,#76470,#76471,#76472,#76473,#76474,
#76475,#76476,#76477,#76478,#76479,#76480,#76481,#76482,#76483,#76484,#76485,
#76486,#76487,#76488,#76489,#76490,#76491,#76492,#76493,#76494,#76495,#76496,
#76497,#76498,#76499,#76500,#76501,#76502,#76503,#76504,#76505,#76506,#76507,
#76508,#76509,#76510,#76511,#76512,#76513,#76514,#76515,#76516,#76517,#76518,
#76519,#76520,#76521,#76522,#76523,#76524,#76525,#76526,#76527,#76528,#76529,
#76530,#76531,#76532,#76533,#76534,#76535,#76536,#76537,#76538,#76539,#76540,
#76541,#76542,#76543,#76544,#76545,#76546,#76547,#76548,#76549,#76550,#76551,
#76552,#76553,#76554,#76555,#76556,#76557,#76558,#76559,#76560,#76561,#76562,
#76563,#76564,#76565,#76566,#76567,#76568,#76569,#76570,#76571,#76572,#76573,
#76574,#76575,#76576,#76577,#76578,#76579,#76580,#76581,#76582,#76583,#76584,
#76585,#76586,#76587,#76588,#76589,#76590,#76591,#76592,#76593,#76594,#76595,
#76596,#76597,#76598,#76599,#76600,#76601,#76602,#76603,#76604,#76605,#76606,
#76607,#76608,#76609,#76610,#76611,#76612,#76613,#76614,#76615,#76616,#76617,
#76618),.UNSPECIFIED.,.F.,.F.,(4,2,2,2,2,2,2,2,2,2,2,2,2,2,2,2,2,2,2,2,
2,2,2,2,2,2,2,2,2,2,2,2,2,2,2,2,2,2,2,2,2,2,2,2,2,2,2,2,2,2,2,2,2,2,2,2,
2,2,2,2,2,2,2,2,2,2,2,2,2,2,2,2,2,2,2,2,2,2,2,2,2,2,2,2,2,2,2,2,2,2,2,2,
2,2,2,2,2,2,2,2,2,2,2,2,2,2,2,2,2,2,2,2,2,2,2,2,2,2,2,2,2,2,2,4),(-1.25986135129038,
-1.24530241304872,-1.18892854063003,-1.17208345698105,-1.1684667484003,
-1.16610265211268,-1.16418885867655,-1.16199670869744,-1.15821041669407,
-1.14196381604285,-1.08448970814712,-1.0795172366509,-1.06353182564182,
-1.06091347502439,-1.05956642115189,-1.05849509636142,-1.05723809537606,
-1.05496301773918,-1.0436118759728,-1.01753002264744,-0.964659587630602,
-0.957756719319972,-0.954888708775274,-0.95309551240865,-0.951134262484446,
-0.948428152624589,-0.942009928704008,-0.913435225488642,-0.862239864547941,
-0.851079020293154,-0.848925868779101,-0.847567519096587,-0.846495407124745,
-0.845246902631221,-0.843010792420016,-0.832315998632985,-0.80872374665589,
-0.752156378070943,-0.745591532409124,-0.743061755128935,-0.741238306696934,
-0.739298245534177,-0.736716176795954,-0.731003276960136,-0.708004592533687,
-0.674986690410184,-0.653922324950132,-0.639428764806459,-0.637099290227801,
-0.635703054238043,-0.634624587936592,-0.633415201032819,-0.631356176608807,
-0.623141284813286,-0.607518365865643,-0.565765413269225,-0.537118824493238,
-0.532954837851641,-0.530451971739961,-0.528517507706292,-0.526428089253623,
-0.523105719214729,-0.512132575251355,-0.494077374872629,-0.443985019031152,
-0.427602851320191,-0.424968414734493,-0.423617988860906,-0.422546549653114,
-0.421292383098954,-0.419029949548998,-0.407894034232583,-0.382647589360761,
-0.328577165374617,-0.321772203085985,-0.318920524702571,-0.317130429035644,
-0.315166827285759,-0.312446895803623,-0.305945402103554,-0.27666548529029,
-0.229654393283906,-0.21545674752028,-0.2129408363912,-0.211630983235744,
-0.210618633622361,-0.210611043586414,-0.210603596973413,-0.21059628534332,
-0.210589100829224,-0.210582036068197,-0.210575084198925,-0.210568238859746,
-0.210561494134435,-0.210554844443709,-0.210548284498576,-0.210541809366055,
-0.210535414439193,-0.210529095285272,-0.210522847770718,-0.210516667985328,
-0.210510552242024,-0.210504496979383,-0.210498498772053,-0.210492554419833,
-0.210486660957257,-0.210480815489451,-0.209218763863868,-0.206836299392488,
-0.193388069173711,-0.157802414423416,-0.113366775909924,-0.109089434563902,
-0.106553571364546,-0.104613969153839,-0.102538903441034,-0.0992814031391307,
-0.0888910015985643,-0.0721524541642749,-0.0417417147298587,-0.00539305727599119,
-0.00193455410719084,-0.000863977557054734,-0.000629065414789221),
 .UNSPECIFIED.);
#803=B_SPLINE_CURVE_WITH_KNOTS('',3,(#76619,#76620,#76621,#76622,#76623,
#76624,#76625,#76626,#76627,#76628,#76629,#76630,#76631,#76632,#76633,#76634),
 .UNSPECIFIED.,.F.,.F.,(4,3,3,3,3,4),(-28.973780262141,-28.9662570488944,
-28.8628842312467,-28.7596459043877,-28.6565264336552,-28.6232428442244),
 .UNSPECIFIED.);
#804=B_SPLINE_CURVE_WITH_KNOTS('',3,(#76639,#76640,#76641,#76642,#76643,
#76644,#76645,#76646,#76647,#76648,#76649,#76650,#76651,#76652,#76653,#76654,
#76655,#76656,#76657,#76658,#76659,#76660,#76661,#76662,#76663,#76664,#76665,
#76666,#76667,#76668,#76669,#76670,#76671,#76672,#76673,#76674,#76675,#76676,
#76677,#76678,#76679,#76680,#76681,#76682,#76683,#76684,#76685,#76686,#76687,
#76688,#76689,#76690,#76691,#76692,#76693,#76694,#76695,#76696,#76697,#76698,
#76699,#76700,#76701,#76702,#76703,#76704,#76705,#76706,#76707,#76708,#76709,
#76710,#76711,#76712,#76713,#76714,#76715,#76716,#76717,#76718,#76719,#76720,
#76721,#76722,#76723,#76724,#76725,#76726,#76727,#76728,#76729,#76730,#76731,
#76732,#76733,#76734,#76735,#76736,#76737,#76738,#76739,#76740,#76741,#76742,
#76743,#76744,#76745,#76746,#76747,#76748,#76749,#76750,#76751,#76752,#76753,
#76754,#76755,#76756,#76757,#76758,#76759,#76760,#76761,#76762,#76763,#76764,
#76765,#76766,#76767,#76768,#76769,#76770,#76771,#76772,#76773,#76774,#76775,
#76776,#76777,#76778,#76779,#76780,#76781,#76782,#76783,#76784,#76785,#76786,
#76787,#76788,#76789,#76790,#76791,#76792,#76793,#76794,#76795,#76796,#76797,
#76798,#76799,#76800,#76801,#76802,#76803,#76804,#76805,#76806,#76807,#76808,
#76809,#76810,#76811,#76812,#76813,#76814,#76815,#76816,#76817,#76818,#76819,
#76820,#76821,#76822,#76823,#76824,#76825,#76826,#76827,#76828,#76829,#76830,
#76831,#76832,#76833,#76834,#76835,#76836,#76837,#76838,#76839,#76840,#76841,
#76842,#76843,#76844,#76845,#76846,#76847,#76848,#76849,#76850,#76851,#76852,
#76853,#76854,#76855,#76856,#76857,#76858,#76859,#76860,#76861,#76862,#76863,
#76864,#76865,#76866,#76867,#76868),.UNSPECIFIED.,.F.,.F.,(4,2,2,2,2,2,
2,2,2,2,2,2,2,2,2,2,2,2,2,2,2,2,2,2,2,2,2,2,2,2,2,2,2,2,2,2,2,2,2,2,2,2,
2,2,2,2,2,2,2,2,2,2,2,2,2,2,2,2,2,2,2,2,2,2,2,2,2,2,2,2,2,2,2,2,2,2,2,2,
2,2,2,2,2,2,2,2,2,2,2,2,2,2,2,2,2,2,2,2,2,2,2,2,2,2,2,2,2,2,2,2,2,2,2,2,
4),(-1.40851932798763,-1.36251967303565,-1.34496387376542,-1.33420949748336,
-1.33091039297545,-1.32882568929973,-1.32688875653648,-1.32432953104823,
-1.31874292200313,-1.31131943588228,-1.29271751926307,-1.24998826934857,
-1.22736039816029,-1.22450822663683,-1.22313156801119,-1.22205771318169,
-1.22082156654236,-1.21864248629277,-1.20883325900351,-1.1599279269835,
-1.12480863003436,-1.12051293205289,-1.11797138246468,-1.11603042508517,
-1.11395681478208,-1.11070767248791,-1.1003953416141,-1.08383154118467,
-1.05096823261267,-1.03714008214105,-1.03049000477807,-1.01501639385347,
-1.01241930562685,-1.01107679765891,-1.01000570146705,-1.00874502699915,
-1.00645320871981,-0.994806460469776,-0.967539938546587,-0.947355528278572,
-0.912847748863482,-0.90856105700415,-0.906022142483153,-0.904081644289435,
-0.90200701681872,-0.898753128330105,-0.888399074567619,-0.871742815617945,
-0.838803247362783,-0.820076463512285,-0.803165902003435,-0.800510799090681,
-0.799155821086824,-0.798083909006519,-0.796832804582979,-0.794584968412347,
-0.783698952920323,-0.759401470361552,-0.703906144516429,-0.697230212082474,
-0.694682827186489,-0.692854664646051,-0.690916922843327,-0.688350416764518,
-0.682722825640793,-0.675230048959998,-0.656373513318399,-0.626172116799537,
-0.603803549513684,-0.590878592279148,-0.588627399430395,-0.587239420040068,
-0.586164651678936,-0.58493632280847,-0.582791965444088,-0.573473453360424,
-0.524286329905296,-0.488922121577425,-0.484624198957251,-0.482082301351664,
-0.480141635517877,-0.478068876837535,-0.474822196268678,-0.464527172285693,
-0.448000188859423,-0.417117631706392,-0.397781521153882,-0.379330553425616,
-0.37658873622334,-0.375234258339661,-0.374162591387321,-0.372911599748906,
-0.370663532494245,-0.360092078763205,-0.336830824961793,-0.28752854758086,
-0.275018187417155,-0.271389981246374,-0.269232925473199,-0.267506777687011,
-0.265182988966667,-0.261107434718789,-0.240159355657591,-0.199117570020485,
-0.167650338839419,-0.164739213826966,-0.163351351009537,-0.162276738228571,
-0.161048660238643,-0.159756431943822,-0.155106585482959,-0.128864138723284,
-0.106990698897584,-0.105541851048307,-0.0751187349318719),
 .UNSPECIFIED.);
#805=B_SPLINE_CURVE_WITH_KNOTS('',3,(#76870,#76871,#76872,#76873,#76874,
#76875,#76876,#76877,#76878,#76879,#76880,#76881,#76882,#76883,#76884,#76885,
#76886,#76887,#76888,#76889,#76890,#76891,#76892,#76893,#76894,#76895,#76896,
#76897,#76898,#76899,#76900,#76901,#76902,#76903,#76904,#76905,#76906,#76907,
#76908,#76909,#76910,#76911,#76912,#76913,#76914,#76915,#76916,#76917,#76918,
#76919,#76920,#76921,#76922,#76923,#76924,#76925,#76926,#76927,#76928,#76929,
#76930,#76931,#76932,#76933,#76934,#76935,#76936,#76937,#76938,#76939,#76940,
#76941,#76942,#76943,#76944,#76945,#76946,#76947,#76948,#76949,#76950,#76951,
#76952,#76953,#76954,#76955,#76956,#76957,#76958,#76959,#76960,#76961,#76962,
#76963,#76964,#76965,#76966,#76967,#76968,#76969,#76970,#76971,#76972,#76973,
#76974,#76975,#76976,#76977,#76978,#76979,#76980,#76981,#76982,#76983,#76984,
#76985,#76986,#76987,#76988,#76989,#76990,#76991,#76992,#76993,#76994,#76995,
#76996,#76997,#76998,#76999,#77000,#77001,#77002,#77003,#77004,#77005,#77006,
#77007,#77008,#77009,#77010,#77011,#77012,#77013,#77014,#77015,#77016,#77017,
#77018,#77019,#77020,#77021,#77022,#77023,#77024,#77025,#77026,#77027,#77028,
#77029,#77030,#77031,#77032,#77033,#77034,#77035,#77036,#77037,#77038,#77039,
#77040,#77041,#77042,#77043,#77044,#77045,#77046,#77047,#77048,#77049,#77050),
 .UNSPECIFIED.,.F.,.F.,(4,3,3,3,3,3,3,3,3,3,3,3,3,3,3,3,3,3,3,3,3,3,3,3,
3,3,3,3,3,3,3,3,3,3,3,3,3,3,3,3,3,3,3,3,3,3,3,3,3,3,3,3,3,3,3,3,3,3,3,3,
4),(-28.6232428442244,-28.520202111683,-28.4171817669707,-28.3141478226609,
-28.2110002317942,-28.1077864632061,-28.0043998658756,-27.9674205989325,
-27.864025861899,-27.7607845797986,-27.6576646144211,-27.5546100462272,
-27.4515868378845,-27.3485609952271,-27.2454282284641,-27.1422391370695,
-27.0388671437029,-26.9685841489706,-26.8651894118466,-26.7619481296554,
-26.658828164187,-26.555773595902,-26.4527503874685,-26.3497245447204,-26.2465917778677,
-26.1434026863838,-26.0400306929296,-25.9697476990087,-25.8663529620658,
-25.7631116800555,-25.659991714767,-25.5569371466611,-25.4539139384057,
-25.3508880958346,-25.2477553291558,-25.1445662378443,-25.0411942445581,
-24.9709112490469,-24.8675165120622,-24.7642752300117,-24.6611552646857,
-24.558100696544,-24.4550774882544,-24.3520516456508,-24.2489188789423,
-24.1457297876027,-24.0423577942913,-23.972074799085,-23.8686800615155,
-23.7654387788772,-23.6623188129617,-23.5592642442299,-23.4562410353503,
-23.3532151921577,-23.2500824248659,-23.1468933329451,-23.0435213390625,
-22.9732383491231,-22.8444301460781,-22.7177283292995,-22.6905949549614),
 .UNSPECIFIED.);
#806=B_SPLINE_CURVE_WITH_KNOTS('',3,(#77051,#77052,#77053,#77054),
 .UNSPECIFIED.,.F.,.F.,(4,4),(-22.6905949549614,-22.3411473213039),
 .UNSPECIFIED.);
#807=B_SPLINE_CURVE_WITH_KNOTS('',3,(#77060,#77061,#77062,#77063,#77064,
#77065,#77066,#77067,#77068,#77069,#77070,#77071,#77072,#77073,#77074,#77075,
#77076,#77077),.UNSPECIFIED.,.F.,.F.,(4,2,2,2,2,2,2,2,4),(-0.0747374607281607,
-0.0441237834881369,-0.0412117014333899,-0.039823612314504,-0.0387489300670153,
-0.0375208908713778,-0.0362287404382341,-0.034250737200593,-0.000628702685456983),
 .UNSPECIFIED.);
#808=B_SPLINE_CURVE_WITH_KNOTS('',3,(#77078,#77079,#77080,#77081,#77082,
#77083,#77084,#77085,#77086,#77087,#77088,#77089,#77090,#77091,#77092,#77093,
#77094,#77095,#77096,#77097,#77098,#77099,#77100,#77101,#77102,#77103,#77104,
#77105,#77106,#77107,#77108,#77109,#77110,#77111,#77112,#77113,#77114,#77115,
#77116,#77117,#77118,#77119,#77120,#77121,#77122,#77123,#77124,#77125,#77126,
#77127,#77128,#77129,#77130,#77131,#77132,#77133,#77134,#77135,#77136,#77137,
#77138,#77139,#77140,#77141,#77142,#77143,#77144,#77145,#77146,#77147,#77148,
#77149,#77150,#77151,#77152,#77153,#77154,#77155,#77156,#77157,#77158,#77159,
#77160,#77161,#77162,#77163,#77164,#77165,#77166,#77167,#77168,#77169,#77170,
#77171,#77172,#77173,#77174,#77175,#77176,#77177,#77178,#77179,#77180,#77181,
#77182,#77183,#77184,#77185,#77186,#77187,#77188,#77189,#77190,#77191,#77192,
#77193,#77194,#77195,#77196,#77197,#77198,#77199,#77200,#77201,#77202,#77203,
#77204,#77205,#77206,#77207,#77208,#77209,#77210,#77211,#77212,#77213,#77214,
#77215,#77216,#77217,#77218,#77219,#77220,#77221,#77222,#77223,#77224,#77225,
#77226,#77227,#77228,#77229,#77230,#77231,#77232,#77233,#77234,#77235,#77236,
#77237,#77238,#77239,#77240,#77241,#77242,#77243,#77244,#77245,#77246,#77247,
#77248,#77249,#77250,#77251,#77252,#77253,#77254,#77255,#77256,#77257,#77258,
#77259,#77260,#77261,#77262,#77263,#77264,#77265,#77266,#77267,#77268,#77269,
#77270,#77271,#77272,#77273,#77274,#77275,#77276,#77277,#77278,#77279,#77280,
#77281,#77282,#77283,#77284,#77285,#77286,#77287,#77288,#77289,#77290,#77291,
#77292,#77293,#77294,#77295),.UNSPECIFIED.,.F.,.F.,(4,2,2,2,2,2,2,2,2,2,
2,2,2,2,2,2,2,2,2,2,2,2,2,2,2,2,2,2,2,2,2,2,2,2,2,2,2,2,2,2,2,2,2,2,2,2,
2,2,2,2,2,2,2,2,2,2,2,2,2,2,2,2,2,2,2,2,2,2,2,2,2,2,2,2,2,2,2,2,2,2,2,2,
2,2,2,2,2,2,2,2,2,2,2,2,2,2,2,2,2,2,2,2,2,2,2,2,2,2,4),(-2.66809505953643,
-2.63761331797238,-2.61110679367198,-2.60494080474704,-2.60227773168817,
-2.60032396047389,-2.59852101349307,-2.59560062553725,-2.58838442381747,
-2.54313761767022,-2.52325627693072,-2.50675385428201,-2.49825766913804,
-2.49621111536066,-2.49497891808633,-2.49390458241747,-2.49252216605694,
-2.48964027606611,-2.45494094605814,-2.41403106020496,-2.3955778961565,
-2.39164569804701,-2.38942139223529,-2.38770157987476,-2.38545882655125,
-2.38154963844257,-2.36550449479325,-2.3555748840692,-2.30780578460153,
-2.29374492971221,-2.28865990585603,-2.28504323286418,-2.28352703141438,
-2.28243359063611,-2.28140957725044,-2.27967633134623,-2.27500874914261,
-2.23339056871752,-2.18625557675148,-2.1806587311454,-2.17809785516819,
-2.17616092327188,-2.17433098820525,-2.17177704313981,-2.16505870553325,
-2.11003460213544,-2.0854500870359,-2.07448670070358,-2.07223421363577,
-2.0709820761646,-2.06991023822469,-2.06855657487153,-2.06581977354791,
-2.04754250227878,-2.02956943461586,-1.99683442078875,-1.97432717202141,
-1.96868039576043,-1.96611017807903,-1.96417168923076,-1.96234433782488,
-1.95980051954979,-1.95314856270812,-1.89742903710516,-1.87330086627225,
-1.86245912606583,-1.86021381154727,-1.85896317051981,-1.85789108033303,
-1.85653513247731,-1.8543902297512,-1.84336766854611,-1.79206530561104,
-1.76340168823991,-1.75697292436754,-1.75426481789332,-1.75230301221034,
-1.75050992491119,-1.7476434204999,-1.74075104945696,-1.68775845932275,
-1.66178343541008,-1.65045820460074,-1.64818443419826,-1.64692761884622,
-1.64585613017212,-1.64450845403046,-1.64188767231965,-1.62586303094119,
-1.62045980395024,-1.60595976788558,-1.57306342699952,-1.5503064766965,
-1.54462578573184,-1.54204923540293,-1.54010966288761,-1.53828399832293,
-1.53574686781244,-1.529138078458,-1.47298732082922,-1.4491376820485,-1.4383709681625,
-1.43613010296641,-1.43488037942495,-1.43380811217426,-1.4324507032515,
-1.42978489789984,-1.41259793855704,-1.40851932798763),.UNSPECIFIED.);
#809=B_SPLINE_CURVE_WITH_KNOTS('',3,(#77297,#77298,#77299,#77300,#77301,
#77302,#77303,#77304,#77305,#77306),.UNSPECIFIED.,.F.,.F.,(4,1,1,1,1,1,
1,4),(-22.3411473213039,-21.9744018991612,-20.9755654491994,-19.9767289992375,
-18.9778925492756,-17.9790560993137,-16.9802196493519,-16.4074096477818),
 .UNSPECIFIED.);
#810=B_SPLINE_CURVE_WITH_KNOTS('',3,(#77307,#77308,#77309,#77310,#77311,
#77312),.UNSPECIFIED.,.F.,.F.,(4,2,4),(-2.66742168182414,-2.60891631380292,
-2.59315594400309),.UNSPECIFIED.);
#811=B_SPLINE_CURVE_WITH_KNOTS('',3,(#77317,#77318,#77319,#77320,#77321,
#77322,#77323,#77324,#77325,#77326,#77327,#77328,#77329,#77330,#77331,#77332,
#77333,#77334,#77335,#77336,#77337,#77338,#77339,#77340,#77341,#77342,#77343,
#77344,#77345,#77346,#77347,#77348,#77349,#77350,#77351,#77352,#77353,#77354,
#77355,#77356,#77357,#77358,#77359,#77360,#77361,#77362,#77363,#77364,#77365,
#77366,#77367,#77368,#77369,#77370,#77371,#77372,#77373,#77374,#77375,#77376,
#77377,#77378,#77379,#77380,#77381,#77382,#77383,#77384,#77385,#77386,#77387,
#77388,#77389,#77390,#77391,#77392,#77393,#77394,#77395,#77396,#77397,#77398,
#77399,#77400,#77401,#77402,#77403,#77404,#77405,#77406,#77407,#77408,#77409,
#77410,#77411,#77412,#77413,#77414,#77415,#77416,#77417,#77418,#77419,#77420,
#77421,#77422,#77423,#77424,#77425,#77426,#77427,#77428,#77429,#77430,#77431,
#77432,#77433,#77434,#77435,#77436,#77437,#77438,#77439,#77440,#77441,#77442,
#77443,#77444,#77445,#77446,#77447,#77448,#77449,#77450,#77451,#77452,#77453,
#77454,#77455,#77456,#77457,#77458,#77459,#77460,#77461,#77462,#77463,#77464,
#77465,#77466,#77467,#77468,#77469,#77470,#77471,#77472,#77473,#77474,#77475,
#77476,#77477,#77478,#77479,#77480,#77481,#77482,#77483,#77484,#77485,#77486,
#77487,#77488,#77489,#77490,#77491,#77492,#77493,#77494,#77495,#77496,#77497,
#77498,#77499,#77500,#77501,#77502,#77503,#77504,#77505,#77506,#77507,#77508,
#77509,#77510,#77511,#77512,#77513,#77514,#77515,#77516,#77517,#77518,#77519,
#77520,#77521,#77522,#77523,#77524,#77525,#77526,#77527,#77528,#77529,#77530,
#77531,#77532,#77533,#77534,#77535,#77536,#77537,#77538,#77539,#77540),
 .UNSPECIFIED.,.F.,.F.,(4,2,2,2,2,2,2,2,2,2,2,2,2,2,2,2,2,2,2,2,2,2,2,2,
2,2,2,2,2,2,2,2,2,2,2,2,2,2,2,2,2,2,2,2,2,2,2,2,2,2,2,2,2,2,2,2,2,2,2,2,
2,2,2,2,2,2,2,2,2,2,2,2,2,2,2,2,2,2,2,2,2,2,2,2,2,2,2,2,2,2,2,2,2,2,2,2,
2,2,2,2,2,2,2,2,2,2,2,2,2,2,2,4),(-1.40821110954925,-1.36481848480488,-1.33376867328224,
-1.31571878383699,-1.3130231632549,-1.31165951849834,-1.31058689517225,
-1.30934198277219,-1.30712267449558,-1.29669950717846,-1.27408620769441,
-1.21596233875948,-1.20957870649379,-1.20707845656185,-1.20526260397841,
-1.20331782760757,-1.20070732681518,-1.19483829682318,-1.17066188426138,
-1.12017878610895,-1.11974730187484,-1.10356130443534,-1.10093436984525,
-1.09958543134425,-1.09851394096311,-1.09725829142831,-1.094989560096,-1.08374965241037,
-1.05810385593581,-1.00460239693588,-0.997748372498273,-0.99488833896926,
-0.993096547627768,-0.991133948949955,-0.988420677784727,-0.981960289021308,
-0.928025358577391,-0.891815848873303,-0.888961284076015,-0.887584262790791,
-0.886510497564794,-0.885274874791088,-0.883097727008738,-0.873313951073665,
-0.824394671026784,-0.789272994150639,-0.784977762009422,-0.782436516651152,
-0.780495808128905,-0.778422479733483,-0.775173812713509,-0.764863274195816,
-0.748302625280135,-0.715444393115923,-0.701701467686459,-0.694857451113974,
-0.694560814745629,-0.689297374813233,-0.678994931801532,-0.67689672763898,
-0.67555521898923,-0.674484310308509,-0.67322314550023,-0.670928611783269,
-0.659228920618754,-0.610479424775481,-0.577268525378623,-0.573005111433949,
-0.570473225836644,-0.568534188769422,-0.566457314082085,-0.563191904701132,
-0.552732891845996,-0.535841971849385,-0.498075526237576,-0.467987735292297,
-0.46507417533318,-0.463685786240215,-0.462611058561022,-0.461383177084474,
-0.459240536492632,-0.44994394434002,-0.431091130978925,-0.387350906491365,
-0.364762305076266,-0.36081450918857,-0.35834922620885,-0.356425700266068,
-0.354297426069673,-0.350799315329481,-0.338078592183232,-0.315779294387565,
-0.265694685127626,-0.255118673220226,-0.253002573467255,-0.251655635915973,
-0.250584471026185,-0.249327735780924,-0.247099073363263,-0.236376527994363,
-0.212617559794168,-0.186546611322787,-0.153396864493389,-0.149134572932028,
-0.146603014355765,-0.144664031112807,-0.142587022380962,-0.13932099922551,
-0.128856559433987,-0.098549695579791,-0.0750525798539899,-0.0747374607281607),
 .UNSPECIFIED.);
#812=B_SPLINE_CURVE_WITH_KNOTS('',3,(#77541,#77542,#77543,#77544,#77545,
#77546,#77547,#77548,#77549,#77550,#77551,#77552,#77553,#77554,#77555,#77556,
#77557,#77558,#77559,#77560,#77561,#77562,#77563,#77564,#77565,#77566,#77567,
#77568,#77569,#77570,#77571,#77572,#77573,#77574,#77575,#77576,#77577,#77578,
#77579,#77580,#77581,#77582,#77583,#77584,#77585,#77586,#77587,#77588,#77589,
#77590,#77591,#77592,#77593,#77594,#77595,#77596,#77597,#77598,#77599,#77600,
#77601,#77602,#77603,#77604,#77605,#77606,#77607,#77608,#77609,#77610,#77611,
#77612,#77613,#77614,#77615,#77616,#77617,#77618,#77619,#77620,#77621,#77622,
#77623,#77624,#77625,#77626,#77627,#77628,#77629,#77630,#77631,#77632,#77633,
#77634,#77635,#77636,#77637,#77638,#77639,#77640,#77641,#77642,#77643,#77644,
#77645,#77646,#77647,#77648,#77649,#77650,#77651,#77652,#77653,#77654,#77655,
#77656,#77657,#77658,#77659,#77660,#77661,#77662,#77663,#77664,#77665,#77666,
#77667,#77668,#77669,#77670,#77671,#77672,#77673,#77674,#77675,#77676,#77677,
#77678,#77679,#77680,#77681,#77682,#77683,#77684,#77685,#77686,#77687,#77688,
#77689,#77690,#77691,#77692,#77693,#77694,#77695,#77696,#77697,#77698,#77699,
#77700,#77701,#77702,#77703,#77704,#77705,#77706,#77707,#77708,#77709,#77710,
#77711,#77712,#77713,#77714,#77715,#77716,#77717,#77718,#77719,#77720,#77721,
#77722,#77723,#77724,#77725,#77726,#77727,#77728,#77729,#77730,#77731,#77732,
#77733,#77734,#77735,#77736,#77737,#77738,#77739,#77740,#77741,#77742,#77743,
#77744,#77745,#77746,#77747,#77748,#77749,#77750,#77751,#77752,#77753,#77754,
#77755,#77756,#77757,#77758,#77759,#77760,#77761,#77762,#77763,#77764,#77765,
#77766,#77767,#77768,#77769,#77770,#77771,#77772,#77773,#77774),
 .UNSPECIFIED.,.F.,.F.,(4,2,2,2,2,2,2,2,2,2,2,2,2,2,2,2,2,2,2,2,2,2,2,2,
2,2,2,2,2,2,2,2,2,2,2,2,2,2,2,2,2,2,2,2,2,2,2,2,2,2,2,2,2,2,2,2,2,2,2,2,
2,2,2,2,2,2,2,2,2,2,2,2,2,2,2,2,2,2,2,2,2,2,2,2,2,2,2,2,2,2,2,2,2,2,2,2,
2,2,2,2,2,2,2,2,2,2,2,2,2,2,2,2,2,2,2,2,4),(-2.59315594400309,-2.59007763676982,
-2.58078446061555,-2.57864196520466,-2.57741405225984,-2.57633922941941,
-2.5749506167247,-2.57203624597322,-2.54226102741123,-2.49162485054994,
-2.48229405620474,-2.47774234381657,-2.47500421303992,-2.47252001085952,
-2.47064395111727,-2.46881749761626,-2.46627614977761,-2.45963793926299,
-2.40382814330879,-2.37977008790781,-2.36894815909931,-2.36670437657868,
-2.36545422852822,-2.36438233142897,-2.36302633592252,-2.36088082150167,
-2.34984370284795,-2.29863021710051,-2.26992299265595,-2.26348965060112,
-2.26078109769207,-2.25881950609727,-2.25702698407049,-2.25416218694483,
-2.24727808144986,-2.19420980221626,-2.16830033475109,-2.15699278329242,
-2.15472036203695,-2.1534639964676,-2.15239272448482,-2.15104510379787,
-2.14842375920586,-2.13238380037999,-2.12707356947599,-2.11250757331232,
-2.07961724050441,-2.06305113666004,-2.05273923107956,-2.0494904567036,
-2.04741714448578,-2.04547651132128,-2.04293545297379,-2.03864076775904,
-2.00353490506159,-1.9546512443564,-1.94486004465277,-1.94268250720782,
-1.94144684564022,-1.94037316729637,-1.93899640786898,-1.93614292224175,
-1.91344482323367,-1.87272167211962,-1.84568035402812,-1.83944843091071,
-1.83677410159091,-1.83481850808743,-1.83301838099935,-1.83011257507762,
-1.82298217100003,-1.77422999705428,-1.73505270581902,-1.73147804015649,
-1.72996902809197,-1.7288768636613,-1.72785087752937,-1.726107663268,-1.72137458018872,
-1.68179593316283,-1.63388990738188,-1.62749310795193,-1.62479053302431,
-1.62282984151228,-1.6210357776119,-1.61816336034547,-1.61123422155785,
-1.55875529170381,-1.53242870486769,-1.52101503587405,-1.51873640302925,
-1.51747861988341,-1.51640744685222,-1.51506158455075,-1.51244823884046,
-1.4965682580066,-1.49069794729026,-1.44666701985389,-1.42810815465924,
-1.41691845401453,-1.41357286054019,-1.41147833468581,-1.40954560736701,
-1.40705404720522,-1.40292854512582,-1.37574265136433,-1.33373204563628,
-1.32763512663023,-1.30978754833016,-1.30709916347252,-1.30573723480036,
-1.30466495358076,-1.30341928440853,-1.30119586157112,-1.29070305630196,
-1.26784056700131,-1.25960928830829),.UNSPECIFIED.);
#813=B_SPLINE_CURVE_WITH_KNOTS('',3,(#77780,#77781,#77782,#77783,#77784,
#77785,#77786,#77787,#77788,#77789,#77790,#77791,#77792,#77793,#77794,#77795,
#77796,#77797,#77798,#77799,#77800,#77801,#77802,#77803,#77804,#77805,#77806,
#77807,#77808,#77809,#77810,#77811,#77812,#77813,#77814,#77815,#77816,#77817,
#77818,#77819,#77820,#77821,#77822,#77823,#77824,#77825,#77826,#77827,#77828,
#77829,#77830,#77831,#77832,#77833,#77834,#77835,#77836,#77837,#77838,#77839,
#77840,#77841,#77842,#77843,#77844,#77845,#77846,#77847,#77848,#77849,#77850,
#77851,#77852,#77853,#77854,#77855,#77856,#77857,#77858,#77859,#77860,#77861,
#77862,#77863,#77864,#77865,#77866,#77867,#77868,#77869,#77870,#77871,#77872,
#77873,#77874,#77875,#77876,#77877,#77878,#77879,#77880,#77881,#77882,#77883,
#77884,#77885),.UNSPECIFIED.,.F.,.F.,(4,3,3,3,3,3,3,3,3,3,3,3,3,3,3,3,3,
3,3,3,3,3,3,3,3,3,3,3,3,3,3,3,3,3,3,4),(-3.49054210138362,-3.38888729762208,
-3.28714621677665,-3.18536357729934,-3.08340265109612,-2.99650934988562,
-2.89298815672403,-2.7896179644128,-2.68636610744677,-2.58317789200706,
-2.48001949625459,-2.37685713986045,-2.27358681231221,-2.17025936584281,
-2.06674931475237,-1.99767289992375,-1.8953694703404,-1.79322009387015,
-1.69118812153633,-1.58921885584019,-1.48727693124249,-1.38532702267508,
-1.28325476444039,-1.1811195089167,-1.07877855598727,-0.998836449961877,
-0.892562814926303,-0.780992463060515,-0.675072152100643,-0.569251436963408,
-0.463502577326272,-0.357797922575414,-0.252080134297595,-0.146357262849723,
-0.0405614307760777,0.),.UNSPECIFIED.);
#814=B_SPLINE_CURVE_WITH_KNOTS('',3,(#77888,#77889,#77890,#77891,#77892,
#77893,#77894,#77895,#77896,#77897,#77898,#77899,#77900,#77901,#77902,#77903,
#77904,#77905,#77906,#77907,#77908,#77909,#77910,#77911,#77912,#77913,#77914,
#77915,#77916,#77917,#77918,#77919,#77920,#77921,#77922,#77923,#77924,#77925,
#77926,#77927,#77928,#77929,#77930,#77931,#77932,#77933,#77934,#77935,#77936,
#77937,#77938,#77939,#77940,#77941,#77942,#77943,#77944,#77945,#77946,#77947,
#77948,#77949,#77950,#77951,#77952,#77953,#77954,#77955,#77956,#77957,#77958,
#77959,#77960,#77961,#77962,#77963,#77964,#77965,#77966,#77967,#77968,#77969,
#77970,#77971,#77972,#77973,#77974,#77975,#77976,#77977,#77978,#77979,#77980,
#77981,#77982,#77983,#77984,#77985,#77986,#77987,#77988,#77989,#77990,#77991,
#77992,#77993,#77994,#77995,#77996,#77997,#77998,#77999,#78000,#78001,#78002,
#78003,#78004,#78005,#78006,#78007,#78008,#78009,#78010,#78011,#78012,#78013,
#78014,#78015,#78016,#78017,#78018,#78019,#78020,#78021,#78022,#78023,#78024,
#78025,#78026,#78027,#78028,#78029,#78030,#78031,#78032,#78033,#78034,#78035,
#78036,#78037,#78038,#78039,#78040,#78041,#78042,#78043,#78044,#78045,#78046,
#78047),.UNSPECIFIED.,.F.,.F.,(4,3,3,3,3,3,3,3,3,3,3,3,3,3,3,3,3,3,3,3,
3,3,3,3,3,3,3,3,3,3,3,3,3,3,3,3,3,3,3,3,3,3,3,3,3,3,3,3,3,3,3,3,3,4),(2.00878451684803,
2.11210413325302,2.21527034106229,2.31831513543173,2.42129472868222,2.52424326611283,
2.62719484999974,2.73025123525842,2.83336461674476,2.93665426095923,2.99650934988563,
3.10008234864184,3.20350565405814,3.30681236784359,3.41005649077515,3.51327177809592,
3.61649194455096,3.7198211439703,3.82320814715696,3.92677824242681,3.9953457998475,
4.09860802522565,4.20171488656681,4.30469822083938,4.40761486436263,4.51049905109401,
4.61338497056926,4.71637738346395,4.8194256584024,4.92265765146998,4.99418224980938,
5.09760362616702,5.20087164810089,5.30401837089659,5.40709969299369,5.51014961192936,
5.61320208205146,5.71636116106699,5.81957642889864,5.92297408622041,5.99301869977126,
6.09643424801845,6.19969680809051,6.30283864671348,6.40591544332069,6.50896120312499,
6.61200988851889,6.71516579043367,6.81837821646031,6.92177360855688,6.99185514973314,
7.09672277111834,7.20139609880503,7.24304101724442),.UNSPECIFIED.);
#815=B_SPLINE_CURVE_WITH_KNOTS('',3,(#78053,#78054,#78055,#78056,#78057,
#78058,#78059,#78060,#78061,#78062,#78063,#78064,#78065,#78066,#78067,#78068,
#78069,#78070,#78071,#78072,#78073,#78074,#78075,#78076,#78077,#78078),
 .UNSPECIFIED.,.F.,.F.,(4,2,2,2,2,2,2,2,2,2,2,2,4),(-0.0747573429482938,
-0.0739377920332611,-0.0616381071463188,-0.0559582138108234,-0.0377856129565647,
-0.0350634467537814,-0.0337175298967136,-0.0326484433152754,-0.0316335720184391,
-0.0303960812896949,-0.0285521141284222,-0.0215327022529327,-0.000655553105070654),
 .UNSPECIFIED.);
#816=B_SPLINE_CURVE_WITH_KNOTS('',3,(#78080,#78081,#78082,#78083,#78084,
#78085,#78086,#78087,#78088,#78089,#78090,#78091,#78092,#78093,#78094,#78095,
#78096,#78097,#78098,#78099,#78100,#78101,#78102,#78103,#78104,#78105,#78106,
#78107,#78108,#78109,#78110,#78111,#78112,#78113,#78114,#78115,#78116,#78117,
#78118,#78119,#78120,#78121,#78122,#78123,#78124,#78125,#78126,#78127,#78128,
#78129,#78130,#78131,#78132,#78133,#78134,#78135,#78136,#78137,#78138,#78139,
#78140,#78141,#78142,#78143,#78144,#78145,#78146,#78147,#78148,#78149,#78150,
#78151,#78152,#78153,#78154,#78155,#78156,#78157,#78158,#78159,#78160,#78161,
#78162,#78163,#78164,#78165,#78166,#78167,#78168,#78169,#78170,#78171,#78172,
#78173,#78174,#78175,#78176,#78177,#78178,#78179,#78180,#78181,#78182,#78183,
#78184,#78185,#78186,#78187,#78188,#78189,#78190,#78191,#78192,#78193,#78194,
#78195,#78196,#78197),.UNSPECIFIED.,.F.,.F.,(4,3,3,3,3,3,3,3,3,3,3,3,3,
3,3,3,3,3,3,3,3,3,3,3,3,3,3,3,3,3,3,3,3,3,3,3,3,3,3,4),(170.955339710339,
171.060905920727,171.162663398586,171.264353088208,171.366010720948,171.467671979619,
171.569433774451,171.671256095252,171.773239609138,171.799869393442,171.903390335715,
172.006760275705,172.110011879462,172.21319984129,172.31635798341,172.419520086533,
172.522790163139,172.626117359596,172.72962716495,172.798705843404,172.901009778732,
173.003159662647,173.105192143119,173.207161917372,173.309104350476,173.411054767032,
173.513127529371,173.615263287867,173.717604736276,173.797542293366,173.903815556868,
174.015385955175,174.121305891971,174.227126233922,174.332874722438,174.438579009226,
174.544296437251,174.650018953138,174.755814439837,174.796378743328),
 .UNSPECIFIED.);
#817=B_SPLINE_CURVE_WITH_KNOTS('',3,(#78201,#78202,#78203,#78204,#78205,
#78206,#78207,#78208,#78209,#78210,#78211,#78212,#78213,#78214,#78215,#78216,
#78217,#78218,#78219,#78220,#78221,#78222,#78223,#78224,#78225,#78226,#78227,
#78228,#78229,#78230,#78231,#78232,#78233,#78234,#78235,#78236,#78237,#78238,
#78239,#78240,#78241,#78242,#78243,#78244,#78245,#78246,#78247,#78248,#78249,
#78250,#78251,#78252,#78253,#78254,#78255,#78256,#78257,#78258,#78259,#78260,
#78261,#78262,#78263,#78264,#78265,#78266,#78267,#78268,#78269,#78270,#78271,
#78272,#78273,#78274,#78275,#78276,#78277,#78278,#78279,#78280,#78281,#78282,
#78283,#78284,#78285,#78286,#78287,#78288,#78289,#78290,#78291,#78292,#78293,
#78294,#78295,#78296,#78297,#78298,#78299,#78300,#78301,#78302,#78303,#78304,
#78305,#78306,#78307,#78308,#78309,#78310,#78311,#78312,#78313,#78314,#78315,
#78316,#78317,#78318,#78319,#78320,#78321,#78322,#78323,#78324,#78325,#78326,
#78327,#78328,#78329,#78330,#78331,#78332,#78333,#78334,#78335,#78336,#78337,
#78338,#78339,#78340,#78341,#78342,#78343,#78344,#78345,#78346,#78347,#78348,
#78349,#78350,#78351,#78352,#78353,#78354,#78355,#78356,#78357,#78358,#78359,
#78360,#78361,#78362,#78363,#78364,#78365,#78366,#78367,#78368,#78369),
 .UNSPECIFIED.,.F.,.F.,(4,3,3,3,3,3,3,3,3,3,3,3,3,3,3,3,3,3,3,3,3,3,3,3,
3,3,3,3,3,3,3,3,3,3,3,3,3,3,3,3,3,3,3,3,3,3,3,3,3,3,3,3,3,3,3,3,4),(-172.787594226732,
-172.684274540723,-172.581108262565,-172.478063397069,-172.375083732247,
-172.272135122901,-172.169183466856,-172.06612700955,-171.963013555969,
-171.859723840347,-171.799869393442,-171.69629638248,-171.592873064501,
-171.489566337677,-171.386322201422,-171.28310690051,-171.179886720216,
-171.076557506667,-170.973170489168,-170.869600379445,-170.801032943481,
-170.697770749322,-170.594663919649,-170.491680617572,-170.388764006554,
-170.285879852593,-170.18299396611,-170.080001586328,-169.976953344622,
-169.873721384615,-169.802196493519,-169.69877510374,-169.595507068251,
-169.492360331767,-169.389278995906,-169.286229063151,-169.183176579175,
-169.080017486348,-168.976802204708,-168.873404533735,-168.803360043557,
-168.699944492016,-168.596681928558,-168.493540086429,-168.390463286242,
-168.28741752279,-168.184368833685,-168.081212927987,-167.978000498131,
-167.874605102172,-167.804523593595,-167.699671782949,-167.594987984343,
-167.490464933024,-167.386036710057,-167.281667200642,-167.203857020092),
 .UNSPECIFIED.);
#818=B_SPLINE_CURVE_WITH_KNOTS('',3,(#78370,#78371,#78372,#78373,#78374,
#78375,#78376,#78377),.UNSPECIFIED.,.F.,.F.,(4,2,2,4),(-2.66731441856907,
-2.64527597576796,-2.59640945473285,-2.59312200712756),.UNSPECIFIED.);
#819=B_SPLINE_CURVE_WITH_KNOTS('',3,(#78382,#78383,#78384,#78385,#78386,
#78387,#78388,#78389,#78390,#78391,#78392,#78393,#78394,#78395,#78396,#78397,
#78398,#78399,#78400,#78401,#78402,#78403,#78404,#78405,#78406,#78407,#78408,
#78409,#78410,#78411,#78412,#78413,#78414,#78415,#78416,#78417,#78418,#78419,
#78420,#78421,#78422,#78423,#78424,#78425,#78426,#78427,#78428,#78429,#78430,
#78431,#78432,#78433,#78434,#78435,#78436,#78437,#78438,#78439,#78440,#78441,
#78442,#78443,#78444,#78445,#78446,#78447,#78448,#78449,#78450,#78451,#78452,
#78453,#78454,#78455,#78456,#78457,#78458,#78459,#78460,#78461,#78462,#78463,
#78464,#78465,#78466,#78467,#78468,#78469,#78470,#78471,#78472,#78473,#78474,
#78475,#78476,#78477,#78478,#78479,#78480,#78481,#78482,#78483,#78484,#78485,
#78486,#78487,#78488,#78489,#78490,#78491,#78492,#78493,#78494,#78495,#78496,
#78497,#78498,#78499,#78500,#78501,#78502,#78503,#78504,#78505,#78506,#78507,
#78508,#78509,#78510,#78511,#78512,#78513,#78514,#78515,#78516,#78517,#78518,
#78519,#78520,#78521,#78522,#78523,#78524,#78525,#78526,#78527,#78528,#78529,
#78530,#78531,#78532,#78533,#78534,#78535,#78536,#78537,#78538,#78539,#78540,
#78541,#78542,#78543,#78544,#78545,#78546,#78547,#78548,#78549,#78550,#78551,
#78552,#78553,#78554,#78555,#78556,#78557,#78558,#78559,#78560,#78561,#78562,
#78563,#78564,#78565,#78566,#78567,#78568,#78569,#78570,#78571,#78572,#78573,
#78574,#78575,#78576,#78577,#78578,#78579,#78580,#78581,#78582,#78583,#78584,
#78585,#78586,#78587,#78588,#78589,#78590,#78591,#78592,#78593,#78594,#78595,
#78596,#78597,#78598,#78599,#78600,#78601,#78602,#78603,#78604,#78605,#78606,
#78607),.UNSPECIFIED.,.F.,.F.,(4,2,2,2,2,2,2,2,2,2,2,2,2,2,2,2,2,2,2,2,
2,2,2,2,2,2,2,2,2,2,2,2,2,2,2,2,2,2,2,2,2,2,2,2,2,2,2,2,2,2,2,2,2,2,2,2,
2,2,2,2,2,2,2,2,2,2,2,2,2,2,2,2,2,2,2,2,2,2,2,2,2,2,2,2,2,2,2,2,2,2,2,2,
2,2,2,2,2,2,2,2,2,2,2,2,2,2,2,2,2,2,2,2,4),(-1.40817978975408,-1.40705404757926,
-1.40292854426818,-1.37574263641332,-1.33373204839412,-1.32763515288138,
-1.30978755251285,-1.3070991662496,-1.30573723699631,-1.30466495537313,
-1.30341928575946,-1.30119586221527,-1.29070305463655,-1.2678405586377,
-1.21011174383134,-1.20367847380292,-1.20117011249373,-1.19935225441946,
-1.1974089632733,-1.19480675666405,-1.18898303420208,-1.16514969212771,
-1.11614974786207,-1.09779133728369,-1.09505199613252,-1.09369780661655,
-1.09262570590498,-1.09137328937515,-1.08912119207965,-1.0781767065768,
-1.05366061664344,-0.998557329887152,-0.991850144205298,-0.989297530946018,
-0.987467664534772,-0.985529988805104,-0.982966731454034,-0.977358991914342,
-0.929074949970343,-0.888723643118344,-0.884011288715337,-0.882271315198972,
-0.881246030966405,-0.880154595229384,-0.878645300073168,-0.875062776341669,
-0.870037648176115,-0.856213770806916,-0.833863019819696,-0.787184849699778,
-0.779989349485372,-0.777074348187559,-0.775273831938472,-0.773322007349834,
-0.770660366843926,-0.764492303368742,-0.737949711517808,-0.698620807892402,
-0.687287567855293,-0.673503613153939,-0.671211219321855,-0.669826486150342,
-0.668750035540309,-0.667534904461336,-0.665449567461102,-0.656908029632808,
-0.640347504304022,-0.59827806430656,-0.5710994647725,-0.566971944369264,
-0.564479121525566,-0.56254537992993,-0.560449714544518,-0.557102195271231,
-0.545904429027561,-0.527329152626984,-0.48480646601045,-0.462028585515264,
-0.459170679768378,-0.457792016141116,-0.456715751535966,-0.455474777491361,
-0.453287201529222,-0.443435529530059,-0.394233009637958,-0.359839125135791,
-0.355551417093985,-0.353009420771898,-0.351065048478533,-0.348984761265523,
-0.345718734049554,-0.335297061988363,-0.318505477259715,-0.25888309088138,
-0.249294095406842,-0.247244764404746,-0.245918148672959,-0.244851109626237,
-0.243841387935879,-0.241868990979533,-0.234450971840351,-0.220917549058247,
-0.192337554262401,-0.147271547762224,-0.143024722909869,-0.140506650841021,
-0.13858064226403,-0.136520200019756,-0.133286033524251,-0.122977060350292,
-0.106384465120274,-0.0845184420639834,-0.0747573429482938),
 .UNSPECIFIED.);
#820=B_SPLINE_CURVE_WITH_KNOTS('',3,(#78608,#78609,#78610,#78611,#78612,
#78613,#78614,#78615,#78616,#78617,#78618,#78619,#78620,#78621,#78622,#78623,
#78624,#78625,#78626,#78627,#78628,#78629,#78630,#78631,#78632,#78633,#78634,
#78635,#78636,#78637,#78638,#78639,#78640,#78641,#78642,#78643,#78644,#78645,
#78646,#78647,#78648,#78649,#78650,#78651,#78652,#78653,#78654,#78655,#78656,
#78657,#78658,#78659,#78660,#78661,#78662,#78663,#78664,#78665,#78666,#78667,
#78668,#78669,#78670,#78671,#78672,#78673,#78674,#78675,#78676,#78677,#78678,
#78679,#78680,#78681,#78682,#78683,#78684,#78685,#78686,#78687,#78688,#78689,
#78690,#78691,#78692,#78693,#78694,#78695,#78696,#78697,#78698,#78699,#78700,
#78701,#78702,#78703,#78704,#78705,#78706,#78707,#78708,#78709,#78710,#78711,
#78712,#78713,#78714,#78715,#78716,#78717,#78718,#78719,#78720,#78721,#78722,
#78723,#78724,#78725,#78726,#78727,#78728,#78729,#78730,#78731,#78732,#78733,
#78734,#78735,#78736,#78737,#78738,#78739,#78740,#78741,#78742,#78743,#78744,
#78745,#78746,#78747,#78748,#78749,#78750,#78751,#78752,#78753,#78754,#78755,
#78756,#78757,#78758,#78759,#78760,#78761,#78762,#78763,#78764,#78765,#78766,
#78767,#78768,#78769,#78770,#78771,#78772,#78773,#78774,#78775,#78776,#78777,
#78778,#78779,#78780,#78781,#78782,#78783,#78784,#78785,#78786,#78787,#78788,
#78789,#78790,#78791,#78792,#78793,#78794,#78795,#78796,#78797,#78798,#78799,
#78800,#78801,#78802,#78803,#78804,#78805,#78806,#78807,#78808,#78809,#78810,
#78811,#78812,#78813,#78814,#78815,#78816,#78817,#78818,#78819,#78820,#78821,
#78822,#78823,#78824,#78825,#78826,#78827,#78828,#78829,#78830,#78831,#78832,
#78833,#78834,#78835,#78836,#78837,#78838,#78839,#78840,#78841),
 .UNSPECIFIED.,.F.,.F.,(4,2,2,2,2,2,2,2,2,2,2,2,2,2,2,2,2,2,2,2,2,2,2,2,
2,2,2,2,2,2,2,2,2,2,2,2,2,2,2,2,2,2,2,2,2,2,2,2,2,2,2,2,2,2,2,2,2,2,2,2,
2,2,2,2,2,2,2,2,2,2,2,2,2,2,2,2,2,2,2,2,2,2,2,2,2,2,2,2,2,2,2,2,2,2,2,2,
2,2,2,2,2,2,2,2,2,2,2,2,2,2,2,2,2,2,2,2,4),(-2.59312200712756,-2.58668664222653,
-2.58451546766303,-2.58328207928504,-2.58220871169981,-2.58083073879879,
-2.57797110541151,-2.54189129239521,-2.50916640239598,-2.49279452047219,
-2.48600086106938,-2.48237496634032,-2.47927467296956,-2.47726818405217,
-2.47532693467477,-2.47278524300085,-2.46848983762896,-2.43346398051266,
-2.38445171182475,-2.37475716805989,-2.37258545116,-2.37135064051444,-2.3702764347687,
-2.36889710847375,-2.36667496243012,-2.35430821956314,-2.30479958419138,
-2.27590736793385,-2.26945213717435,-2.26673989329341,-2.26477762736604,
-2.26298586221718,-2.26012525570338,-2.2532666535172,-2.19985319559646,
-2.17417358948347,-2.16292484364099,-2.16065595593984,-2.15940043029352,
-2.15832922288703,-2.15698085418778,-2.15435556021802,-2.13819906501921,
-2.09170618377056,-2.06374275210145,-2.05739900543972,-2.05470588691118,
-2.05274730735861,-2.05095189213046,-2.04807012337105,-2.04108147920287,
-1.98950767075604,-1.96254154867394,-1.95096912120203,-1.94868193553589,
-1.94742248507266,-1.94635153844779,-1.94500812553222,-1.94240635973622,
-1.92681824445236,-1.92033667215102,-1.90643681031755,-1.87355463531687,
-1.85699769932198,-1.84668979822785,-1.84344136769288,-1.84136805127564,
-1.83942725599496,-1.83688575556629,-1.8325898016913,-1.79739244058602,
-1.74815277494505,-1.73876782088624,-1.73661853308056,-1.73538902213904,
-1.73431434234439,-1.73292790728223,-1.73002499827752,-1.69795902725883,
-1.66507249079384,-1.64624588722739,-1.63876175178362,-1.63313965414123,
-1.63057416151338,-1.62863657680158,-1.62680811852904,-1.62425960748694,
-1.61757631709381,-1.56218589452321,-1.53784546862036,-1.52694726338165,
-1.52469875308918,-1.52344751702551,-1.52237564722492,-1.52102091575383,
-1.51836687517718,-1.5014851364578,-1.48269888091522,-1.44973485971465,
-1.4330826113428,-1.42273146978707,-1.41947796277252,-1.41740345786126,
-1.41546299044009,-1.41292399686323,-1.40863693737991,-1.3648787607464,
-1.33382957462007,-1.31578004819068,-1.3130844819512,-1.31172086469994,
-1.31064826301276,-1.30940337573073,-1.30718411226304,-1.29676115595744,
-1.27414831556036,-1.2596648285931),.UNSPECIFIED.);
#821=B_SPLINE_CURVE_WITH_KNOTS('',3,(#78847,#78848,#78849,#78850),
 .UNSPECIFIED.,.F.,.F.,(4,4),(158.039785789814,158.388969095546),
 .UNSPECIFIED.);
#822=B_SPLINE_CURVE_WITH_KNOTS('',3,(#78851,#78852,#78853,#78854,#78855,
#78856,#78857,#78858,#78859,#78860,#78861,#78862,#78863,#78864,#78865,#78866,
#78867,#78868,#78869,#78870,#78871,#78872,#78873,#78874,#78875,#78876,#78877,
#78878,#78879,#78880,#78881,#78882,#78883,#78884,#78885,#78886,#78887,#78888,
#78889,#78890,#78891,#78892,#78893,#78894,#78895,#78896,#78897,#78898,#78899,
#78900,#78901,#78902,#78903,#78904,#78905,#78906,#78907,#78908,#78909,#78910,
#78911,#78912,#78913,#78914,#78915,#78916,#78917,#78918,#78919,#78920,#78921,
#78922,#78923,#78924,#78925,#78926,#78927,#78928,#78929,#78930,#78931,#78932,
#78933,#78934,#78935,#78936,#78937,#78938,#78939,#78940,#78941,#78942,#78943,
#78944,#78945,#78946,#78947,#78948,#78949,#78950,#78951,#78952,#78953,#78954,
#78955,#78956,#78957,#78958,#78959,#78960,#78961,#78962,#78963,#78964,#78965,
#78966,#78967,#78968,#78969,#78970,#78971,#78972,#78973,#78974,#78975,#78976,
#78977,#78978,#78979,#78980,#78981,#78982,#78983,#78984,#78985,#78986,#78987,
#78988,#78989,#78990,#78991,#78992,#78993,#78994,#78995,#78996,#78997,#78998,
#78999,#79000,#79001,#79002,#79003,#79004,#79005,#79006,#79007,#79008,#79009,
#79010,#79011,#79012,#79013,#79014,#79015,#79016,#79017,#79018,#79019,#79020,
#79021,#79022,#79023,#79024,#79025,#79026,#79027,#79028,#79029,#79030,#79031,
#79032,#79033,#79034,#79035,#79036,#79037,#79038,#79039,#79040,#79041,#79042,
#79043,#79044,#79045,#79046,#79047,#79048,#79049,#79050,#79051,#79052,#79053,
#79054,#79055,#79056,#79057,#79058,#79059,#79060),.UNSPECIFIED.,.F.,.F.,
(4,2,2,2,2,2,2,2,2,2,2,2,2,2,2,2,2,2,2,2,2,2,2,2,2,2,2,2,2,2,2,2,2,2,2,
2,2,2,2,2,2,2,2,2,2,2,2,2,2,2,2,2,2,2,2,2,2,2,2,2,2,2,2,2,2,2,2,2,2,2,2,
2,2,2,2,2,2,2,2,2,2,2,2,2,2,2,2,2,2,2,2,2,2,2,2,2,2,2,2,2,2,2,2,2,4),(-2.66742162310756,
-2.60891625458958,-2.59007756301913,-2.5807843811516,-2.57864188477314,
-2.57741397132789,-2.57633914807995,-2.57495053489239,-2.57203616322235,
-2.54225915154028,-2.491618626458,-2.48229125892587,-2.47774074752514,-2.47500310992017,
-2.47251926151665,-2.47064325906592,-2.46881669433059,-2.46627492665722,
-2.45963404079168,-2.40385030414874,-2.37977515805284,-2.36894861844136,
-2.36670455611624,-2.36545434690764,-2.36438245579056,-2.36302654277748,
-2.36088129925783,-2.34984855699457,-2.29862620291396,-2.26992235611622,
-2.26348941602719,-2.2607809307943,-2.2588193513631,-2.25702681510704,-2.25416194012492,
-2.24727736198246,-2.19421525541888,-2.16830149607979,-2.1569928499235,
-2.15472036560436,-2.15346398626832,-2.1523927153326,-2.15104511224504,
-2.1484238498383,-2.13238520146658,-2.12706656171519,-2.11250730991782,
-2.07961705504466,-2.06305104502602,-2.0527391816087,-2.04949041180652,
-2.04741710040982,-2.04547646653824,-2.04293540513378,-2.038640709969,-2.00353412150858,
-1.95464821348685,-1.94485967236405,-1.94268231602897,-1.94144669416129,
-1.9403730099634,-1.93899619029812,-1.93614239862554,-1.91343183992003,
-1.87271682037077,-1.84567960098941,-1.83944818222358,-1.83677393968413,
-1.83481836125248,-1.83301821422818,-1.83011230107754,-1.82298125839401,
-1.77424539366048,-1.73505279865914,-1.73147806163526,-1.72996903731451,
-1.7288768707321,-1.72785088802919,-1.72610769100588,-1.72137472109072,
-1.68178295833899,-1.63388986388747,-1.62749309178188,-1.62479052149567,
-1.62282983083475,-1.62103576597798,-1.61816334339362,-1.61123417222076,
-1.55875570359449,-1.53242879584004,-1.52101504596968,-1.51873640844595,
-1.51747862424396,-1.51640745109487,-1.51506158968022,-1.51244824903978,
-1.49656849145573,-1.49069768702886,-1.44666703851389,-1.4281081634151,
-1.41691845775053,-1.41357286304999,-1.4114783364764,-1.40954560852309,
-1.40817978975408),.UNSPECIFIED.);
#823=B_SPLINE_CURVE_WITH_KNOTS('',3,(#79062,#79063,#79064,#79065,#79066,
#79067,#79068,#79069,#79070,#79071,#79072,#79073,#79074,#79075,#79076,#79077,
#79078,#79079,#79080,#79081,#79082,#79083,#79084,#79085,#79086,#79087,#79088,
#79089,#79090,#79091,#79092,#79093,#79094,#79095,#79096,#79097,#79098,#79099,
#79100,#79101,#79102,#79103,#79104,#79105,#79106,#79107,#79108,#79109,#79110,
#79111,#79112,#79113,#79114,#79115,#79116,#79117,#79118,#79119,#79120,#79121,
#79122,#79123,#79124,#79125,#79126,#79127,#79128,#79129,#79130,#79131,#79132,
#79133,#79134,#79135,#79136,#79137,#79138,#79139,#79140,#79141,#79142,#79143,
#79144,#79145,#79146,#79147,#79148,#79149,#79150,#79151,#79152,#79153,#79154,
#79155,#79156,#79157,#79158,#79159,#79160,#79161,#79162,#79163,#79164,#79165,
#79166,#79167,#79168,#79169,#79170,#79171,#79172,#79173,#79174,#79175,#79176,
#79177,#79178,#79179,#79180,#79181,#79182,#79183,#79184,#79185,#79186,#79187,
#79188,#79189,#79190,#79191,#79192,#79193,#79194,#79195,#79196,#79197,#79198,
#79199,#79200,#79201,#79202,#79203,#79204,#79205,#79206,#79207,#79208,#79209,
#79210,#79211,#79212,#79213,#79214,#79215,#79216,#79217,#79218,#79219,#79220,
#79221,#79222,#79223,#79224,#79225,#79226,#79227,#79228,#79229,#79230,#79231,
#79232,#79233,#79234,#79235,#79236,#79237,#79238,#79239,#79240,#79241,#79242,
#79243,#79244,#79245,#79246,#79247,#79248,#79249,#79250,#79251,#79252,#79253,
#79254,#79255,#79256,#79257,#79258,#79259,#79260,#79261,#79262,#79263,#79264,
#79265,#79266,#79267,#79268,#79269,#79270,#79271,#79272,#79273,#79274,#79275,
#79276,#79277,#79278,#79279,#79280,#79281),.UNSPECIFIED.,.F.,.F.,(4,2,2,
2,2,2,2,2,2,2,2,2,2,2,2,2,2,2,2,2,2,2,2,2,2,2,2,2,2,2,2,2,2,2,2,2,2,2,2,
2,2,2,2,2,2,2,2,2,2,2,2,2,2,2,2,2,2,2,2,2,2,2,2,2,2,2,2,2,2,2,2,2,2,2,2,
2,2,2,2,2,2,2,2,2,2,2,2,2,2,2,2,2,2,2,2,2,2,2,2,2,2,2,2,2,2,2,2,2,2,4),
(-1.2596648285931,-1.2160256105695,-1.2096421076692,-1.20714190826177,-1.20532609232373,
-1.20338135515468,-1.20077090690376,-1.19490199470179,-1.17072606542606,
-1.12024397579635,-1.11981226220589,-1.10362682585641,-1.1009999536592,
-1.09965104438236,-1.09857957574208,-1.09732394998322,-1.09505525728509,
-1.08381545338579,-1.05816969650078,-1.00467000549561,-0.997816063283325,
-0.994956078215463,-0.993164321344302,-0.991201763735631,-0.9884885554406,
-0.982028345407357,-0.928096146003009,-0.891885568568339,-0.889031116345708,
-0.887654133636997,-0.886580391096139,-0.885344786076734,-0.883167649594423,
-0.873383593198826,-0.824465702367648,-0.789344862391968,-0.785049718549043,
-0.782508524928635,-0.78056785562871,-0.778494568855833,-0.775245966469818,
-0.764935628182494,-0.748375296264231,-0.715517712106479,-0.701773749074622,
-0.694932998493534,-0.69464545217534,-0.689556244560843,-0.679089800365006,
-0.676980766915887,-0.675635951791255,-0.6745648624677,-0.673306342658668,
-0.671023941274004,-0.659541239303526,-0.632935074326423,-0.58081796313325,
-0.573862309108464,-0.570985764847464,-0.569191131977569,-0.567231433180628,
-0.564533168175351,-0.558160381320284,-0.529962513252371,-0.48202816084319,
-0.479449715698858,-0.467293909964139,-0.465083541170018,-0.463707902381071,
-0.462634409181775,-0.461398188828441,-0.459217800486224,-0.44938304164365,
-0.400515271221216,-0.365413816321955,-0.361119437563833,-0.358578636710422,
-0.356638232829069,-0.354565196109159,-0.351316915525819,-0.341007007627579,
-0.324446804163342,-0.269351910025381,-0.255460701928919,-0.253161866437407,
-0.251774646689025,-0.250697368696635,-0.249482829523745,-0.247442360045852,
-0.239362587541947,-0.224064932594649,-0.19411672439862,-0.189603855941387,
-0.15347084623078,-0.148747386689599,-0.146324297302805,-0.144405427518325,
-0.142252821210166,-0.138645212087007,-0.124695234879609,-0.0975109104562382,
-0.0749657652856314,-0.0441240231168734,-0.041211786302814,-0.0398236671605482,
-0.0387489818054857,-0.0375209615861949,-0.0362288381666934,-0.0342509000805209,
-0.000628703125059541),.UNSPECIFIED.);
#824=B_SPLINE_CURVE_WITH_KNOTS('',3,(#79282,#79283,#79284,#79285,#79286,
#79287,#79288,#79289,#79290,#79291,#79292,#79293,#79294,#79295,#79296,#79297,
#79298,#79299),.UNSPECIFIED.,.F.,.F.,(4,2,2,2,2,2,2,2,4),(-2.66818930628053,
-2.63771571888677,-2.61120086164018,-2.60503375764702,-2.60237044757543,
-2.60041659460138,-2.59861363688443,-2.59569337617825,-2.59370492657453),
 .UNSPECIFIED.);
#825=B_SPLINE_CURVE_WITH_KNOTS('',3,(#79305,#79306,#79307,#79308,#79309,
#79310,#79311,#79312,#79313,#79314,#79315,#79316,#79317),.UNSPECIFIED.,
 .F.,.F.,(4,3,3,3,4),(151.755345396751,151.823140394205,151.951948597258,
152.078650414045,152.105783788367),.UNSPECIFIED.);
#826=B_SPLINE_CURVE_WITH_KNOTS('',3,(#79318,#79319,#79320,#79321,#79322,
#79323,#79324,#79325,#79326,#79327),.UNSPECIFIED.,.F.,.F.,(4,1,1,1,1,1,
1,4),(152.105783788367,152.821976844167,153.820813294129,154.819649744091,
155.818486194052,156.817322644014,157.816159093976,158.039785789814),
 .UNSPECIFIED.);
#827=B_SPLINE_CURVE_WITH_KNOTS('',3,(#79328,#79329,#79330,#79331,#79332,
#79333,#79334,#79335,#79336,#79337,#79338,#79339,#79340,#79341,#79342,#79343,
#79344,#79345,#79346,#79347,#79348,#79349,#79350,#79351,#79352,#79353,#79354,
#79355,#79356,#79357,#79358,#79359,#79360,#79361,#79362,#79363,#79364,#79365,
#79366,#79367,#79368,#79369,#79370,#79371,#79372,#79373,#79374,#79375,#79376,
#79377,#79378,#79379,#79380,#79381,#79382,#79383,#79384,#79385,#79386,#79387,
#79388,#79389,#79390,#79391,#79392,#79393,#79394,#79395,#79396,#79397,#79398,
#79399,#79400,#79401,#79402,#79403,#79404,#79405,#79406,#79407,#79408,#79409,
#79410,#79411,#79412,#79413,#79414,#79415,#79416,#79417,#79418,#79419,#79420,
#79421,#79422,#79423,#79424,#79425,#79426,#79427,#79428,#79429,#79430,#79431,
#79432,#79433,#79434,#79435,#79436,#79437,#79438,#79439,#79440,#79441,#79442,
#79443,#79444,#79445,#79446,#79447,#79448,#79449,#79450,#79451,#79452,#79453,
#79454,#79455,#79456,#79457,#79458,#79459,#79460,#79461,#79462,#79463,#79464,
#79465,#79466,#79467,#79468,#79469,#79470,#79471,#79472,#79473,#79474,#79475,
#79476,#79477,#79478,#79479,#79480,#79481,#79482,#79483,#79484,#79485,#79486,
#79487,#79488,#79489,#79490,#79491,#79492,#79493,#79494,#79495,#79496,#79497,
#79498,#79499,#79500,#79501,#79502,#79503,#79504,#79505,#79506,#79507,#79508,
#79509,#79510,#79511,#79512,#79513,#79514,#79515,#79516,#79517,#79518,#79519,
#79520,#79521,#79522,#79523,#79524,#79525,#79526,#79527,#79528,#79529,#79530,
#79531,#79532,#79533,#79534,#79535,#79536,#79537,#79538,#79539,#79540,#79541,
#79542,#79543,#79544,#79545,#79546,#79547,#79548,#79549,#79550,#79551,#79552,
#79553,#79554,#79555),.UNSPECIFIED.,.F.,.F.,(4,2,2,2,2,2,2,2,2,2,2,2,2,
2,2,2,2,2,2,2,2,2,2,2,2,2,2,2,2,2,2,2,2,2,2,2,2,2,2,2,2,2,2,2,2,2,2,2,2,
2,2,2,2,2,2,2,2,2,2,2,2,2,2,2,2,2,2,2,2,2,2,2,2,2,2,2,2,2,2,2,2,2,2,2,2,
2,2,2,2,2,2,2,2,2,2,2,2,2,2,2,2,2,2,2,2,2,2,2,2,2,2,2,2,4),(-2.59370492657453,
-2.58847820404563,-2.54309870392059,-2.52300656285645,-2.50674703366011,
-2.49833489705349,-2.49628759775399,-2.49505880127077,-2.49398388929921,
-2.4925960638836,-2.49034578019742,-2.47744469912304,-2.47491956480728,
-2.4706232200629,-2.43000257545183,-2.39666005130046,-2.39214965110867,
-2.38980199149159,-2.38788898195058,-2.38568383373875,-2.38193830658902,
-2.36780631242021,-2.35546526585911,-2.30760509909679,-2.29374245395045,
-2.28870603116317,-2.28511616897621,-2.28360448725736,-2.28251180258687,
-2.28148650553305,-2.27974684899653,-2.27503731979819,-2.23463373138629,
-2.18635069491183,-2.18074307863355,-2.17818014888768,-2.17624284221069,
-2.17441342314041,-2.17186160147031,-2.16515753442451,-2.10997738320941,
-2.0854945172373,-2.07455798185226,-2.07230703406436,-2.07105520034447,
-2.06998328344636,-2.06862908631448,-2.06588979216297,-2.04753865035993,
-2.02964535200168,-1.99690771674675,-1.97439756890853,-1.96875029208805,
-1.96617991876962,-1.96424134195001,-1.96241392924407,-1.95987006037063,
-1.95321817931557,-1.89749282082125,-1.87336596542637,-1.86252439907145,
-1.86027902910937,-1.85902834440211,-1.85795620888598,-1.85660019358752,
-1.85445516523925,-1.84343155678569,-1.79212673046656,-1.76346276898746,
-1.7570338390636,-1.7543256372076,-1.75236375319437,-1.75057058794909,-1.74770394510717,
-1.74081116961503,-1.6878179276519,-1.66184074592123,-1.65051477013927,
-1.64824088959472,-1.64698401865768,-1.64591248581013,-1.64456475820447,
-1.64194388845335,-1.62591893105205,-1.62051388797226,-1.60601441996286,
-1.57311672598438,-1.55035885106369,-1.54467792700712,-1.54210127023863,
-1.54016161730759,-1.53833587683694,-1.53579864049959,-1.52918957349922,
-1.4730365142259,-1.4491858646681,-1.43841869818796,-1.43617773964232,-1.43492796416028,
-1.43385565241863,-1.4324981872711,-1.42983227179874,-1.41264461335246,
-1.36256425545815,-1.34500772461246,-1.33425290066633,-1.33095365909261,
-1.3288688688674,-1.3269318557328,-1.32437252411668,-1.31878568366601,-1.31136189021472,
-1.29275920440411,-1.2599124547823),.UNSPECIFIED.);
#828=B_SPLINE_CURVE_WITH_KNOTS('',3,(#79561,#79562,#79563,#79564,#79565,
#79566,#79567,#79568,#79569,#79570,#79571,#79572,#79573,#79574),
 .UNSPECIFIED.,.F.,.F.,(4,2,2,2,2,2,4),(-0.0749176319822858,-0.0721945338621709,
-0.0417574974960581,-0.00539334313703774,-0.00193462587292075,-0.000864005353919265,
-0.000629064028114969),.UNSPECIFIED.);
#829=B_SPLINE_CURVE_WITH_KNOTS('',3,(#79575,#79576,#79577,#79578,#79579,
#79580,#79581,#79582,#79583,#79584,#79585,#79586,#79587,#79588,#79589,#79590,
#79591,#79592,#79593,#79594,#79595,#79596,#79597,#79598,#79599,#79600,#79601,
#79602,#79603,#79604,#79605,#79606,#79607,#79608,#79609,#79610,#79611,#79612,
#79613,#79614,#79615,#79616,#79617,#79618,#79619,#79620,#79621,#79622,#79623,
#79624,#79625,#79626,#79627,#79628,#79629,#79630,#79631,#79632,#79633,#79634,
#79635,#79636,#79637,#79638,#79639,#79640,#79641,#79642,#79643,#79644,#79645,
#79646,#79647,#79648,#79649,#79650,#79651,#79652,#79653,#79654,#79655,#79656,
#79657,#79658,#79659,#79660,#79661,#79662,#79663,#79664,#79665,#79666,#79667,
#79668,#79669,#79670,#79671,#79672,#79673,#79674,#79675,#79676,#79677,#79678,
#79679,#79680,#79681,#79682,#79683,#79684,#79685,#79686,#79687,#79688,#79689,
#79690,#79691,#79692,#79693,#79694,#79695,#79696,#79697,#79698,#79699,#79700,
#79701,#79702,#79703,#79704,#79705,#79706,#79707,#79708,#79709,#79710,#79711,
#79712,#79713,#79714,#79715,#79716,#79717,#79718,#79719,#79720,#79721,#79722,
#79723,#79724,#79725,#79726,#79727,#79728,#79729,#79730,#79731,#79732,#79733,
#79734,#79735,#79736,#79737,#79738,#79739,#79740,#79741,#79742,#79743,#79744,
#79745,#79746,#79747,#79748,#79749,#79750,#79751,#79752,#79753,#79754,#79755),
 .UNSPECIFIED.,.F.,.F.,(4,3,3,3,3,3,3,3,3,3,3,3,3,3,3,3,3,3,3,3,3,3,3,3,
3,3,3,3,3,3,3,3,3,3,3,3,3,3,3,3,3,3,3,3,3,3,3,3,3,3,3,3,3,3,3,3,3,3,3,3,
4),(145.822598481187,145.830121694434,145.93351643147,146.036757713572,
146.139877678953,146.24293224715,146.345955455495,146.448981298156,146.552114064923,
146.655303156321,146.758675149692,146.828958144396,146.932352881429,147.03559416353,
147.138714128907,147.241768697101,147.344791905443,147.4478177481,147.550950514863,
147.654139606258,147.757511599624,147.827794594357,147.931189331481,148.034430613671,
148.137550579139,148.240605147424,148.343628355857,148.446654198605,148.549786965457,
148.652976056941,148.756348050395,148.826631044319,148.930025781262,149.033267063273,
149.136387028562,149.239441596669,149.342464804925,149.445490647496,149.548623414176,
149.651812505488,149.755184498775,149.825467494281,149.928862231266,150.032103513317,
150.135223478643,150.238278046785,150.341301255075,150.444327097679,150.547459864388,
150.650648955728,150.754020949039,150.824303944243,150.927703487107,151.031158725813,
151.134277032367,151.237328082884,151.340345916045,151.444095786221,151.547200179175,
151.651272787963,151.755345396751),.UNSPECIFIED.);
#830=B_SPLINE_CURVE_WITH_KNOTS('',3,(#79757,#79758,#79759,#79760,#79761,
#79762,#79763,#79764,#79765,#79766,#79767,#79768,#79769,#79770,#79771,#79772,
#79773,#79774,#79775,#79776,#79777,#79778,#79779,#79780,#79781,#79782,#79783,
#79784,#79785,#79786,#79787,#79788,#79789,#79790,#79791,#79792,#79793,#79794,
#79795,#79796,#79797,#79798,#79799,#79800,#79801,#79802,#79803,#79804,#79805,
#79806,#79807,#79808,#79809,#79810,#79811,#79812,#79813,#79814,#79815,#79816,
#79817,#79818,#79819,#79820,#79821,#79822,#79823,#79824,#79825,#79826,#79827,
#79828,#79829,#79830,#79831,#79832,#79833,#79834,#79835,#79836,#79837,#79838,
#79839,#79840,#79841,#79842,#79843,#79844,#79845,#79846,#79847,#79848,#79849,
#79850,#79851,#79852,#79853,#79854,#79855,#79856,#79857,#79858,#79859,#79860,
#79861,#79862,#79863,#79864,#79865,#79866,#79867,#79868,#79869,#79870,#79871,
#79872,#79873,#79874,#79875,#79876,#79877,#79878,#79879,#79880,#79881,#79882,
#79883,#79884,#79885,#79886,#79887,#79888,#79889,#79890,#79891,#79892,#79893,
#79894,#79895,#79896,#79897,#79898,#79899,#79900,#79901,#79902,#79903,#79904,
#79905,#79906,#79907,#79908,#79909,#79910,#79911,#79912,#79913,#79914,#79915,
#79916,#79917,#79918,#79919,#79920,#79921,#79922,#79923,#79924,#79925,#79926,
#79927,#79928,#79929,#79930,#79931,#79932,#79933,#79934,#79935,#79936,#79937,
#79938,#79939,#79940,#79941,#79942,#79943,#79944,#79945,#79946,#79947,#79948,
#79949,#79950,#79951,#79952,#79953,#79954,#79955,#79956,#79957,#79958,#79959,
#79960,#79961,#79962,#79963,#79964,#79965,#79966,#79967,#79968,#79969,#79970,
#79971,#79972,#79973,#79974,#79975,#79976,#79977,#79978,#79979,#79980),
 .UNSPECIFIED.,.F.,.F.,(4,2,2,2,2,2,2,2,2,2,2,2,2,2,2,2,2,2,2,2,2,2,2,2,
2,2,2,2,2,2,2,2,2,2,2,2,2,2,2,2,2,2,2,2,2,2,2,2,2,2,2,2,2,2,2,2,2,2,2,2,
2,2,2,2,2,2,2,2,2,2,2,2,2,2,2,2,2,2,2,2,2,2,2,2,2,2,2,2,2,2,2,2,2,2,2,2,
2,2,2,2,2,2,2,2,2,2,2,2,2,2,2,4),(-1.2599124547823,-1.25002807386397,-1.22739935917188,
-1.2245470716002,-1.22317035629757,-1.22209645694531,-1.22086025870375,
-1.21868108665142,-1.20887143217979,-1.1599640872171,-1.12484333499143,
-1.12054745872809,-1.1180058036613,-1.1160647657301,-1.11399106937169,-1.11074179224174,
-1.10042903347153,-1.08386454585292,-1.05099987303016,-1.03717122403354,
-1.03052069631196,-1.0150465323747,-1.01244934016723,-1.01110677730609,
-1.01003563671185,-1.00877490927762,-1.00648299290409,-0.994835707568061,
-0.967567834981807,-0.947382712475257,-0.912873645829924,-0.90858677832834,
-0.906047759094729,-0.904107180475675,-0.902032466638724,-0.898778441893425,
-0.888423947808562,-0.871766974134913,-0.838826018849427,-0.820097685720636,
-0.803187199701922,-0.800532015826634,-0.799176987846143,-0.798105031739481,
-0.79685387076215,-0.794605920055246,-0.783719099969251,-0.759419292369503,
-0.703923646265877,-0.697247242300925,-0.694699721534836,-0.69287147513404,
-0.690933656972484,-0.688367071008456,-0.682739390828016,-0.675246546493855,
-0.656390119530333,-0.626116411631464,-0.603702869700675,-0.59088098658125,
-0.588635025015686,-0.587248588310373,-0.586173941024472,-0.584944548023931,
-0.582795509189763,-0.57341270182101,-0.524152073686013,-0.488926964416472,
-0.484630607594345,-0.482089109817155,-0.480148446279506,-0.478075396397384,
-0.47482764680899,-0.464524072357827,-0.447978458492938,-0.41710515898568,
-0.397464619463284,-0.37931813610327,-0.37661976383513,-0.375255693963338,
-0.374183237474751,-0.372939096883373,-0.370722545647898,-0.360688865171072,
-0.312016982578369,-0.2769834080816,-0.272689986555764,-0.270149477532661,
-0.268209138396986,-0.266136017507042,-0.262887284792429,-0.25276849119224,
-0.23654606782421,-0.198322585414324,-0.167652355293061,-0.164739955608835,
-0.16335184523917,-0.162277206557913,-0.161049284407586,-0.159757278089317,
-0.155110106861215,-0.128864893942761,-0.106990886563457,-0.105560230878355,
-0.0651104974991618,-0.0603738601647401,-0.0579480736937648,-0.0560290637456423,
-0.0538783940964652,-0.0516516915055142,-0.0483298719236029,-0.00062898557017253),
 .UNSPECIFIED.);
#831=B_SPLINE_CURVE_WITH_KNOTS('',3,(#79981,#79982,#79983,#79984,#79985,
#79986,#79987,#79988,#79989,#79990,#79991,#79992,#79993,#79994,#79995,#79996,
#79997,#79998,#79999,#80000),.UNSPECIFIED.,.F.,.F.,(4,2,2,2,2,2,2,2,2,4),
(-2.66773620090402,-2.62477875133751,-2.6218447624627,-2.62016197467351,
-2.61865699930487,-2.61756533538186,-2.61653793993882,-2.6147881679525,
-2.61001317239784,-2.59360340364756),.UNSPECIFIED.);
#832=B_SPLINE_CURVE_WITH_KNOTS('',3,(#80005,#80006,#80007,#80008,#80009,
#80010,#80011,#80012,#80013,#80014,#80015,#80016,#80017,#80018,#80019,#80020,
#80021,#80022,#80023,#80024,#80025,#80026,#80027,#80028,#80029,#80030,#80031,
#80032,#80033,#80034,#80035,#80036,#80037,#80038,#80039,#80040,#80041,#80042,
#80043,#80044,#80045,#80046,#80047,#80048,#80049,#80050,#80051,#80052,#80053,
#80054,#80055,#80056,#80057,#80058,#80059,#80060,#80061,#80062,#80063,#80064,
#80065,#80066,#80067,#80068,#80069,#80070,#80071,#80072,#80073,#80074,#80075,
#80076,#80077,#80078,#80079,#80080,#80081,#80082,#80083,#80084,#80085,#80086,
#80087,#80088,#80089,#80090,#80091,#80092,#80093,#80094,#80095,#80096,#80097,
#80098,#80099,#80100,#80101,#80102,#80103,#80104,#80105,#80106,#80107,#80108,
#80109,#80110,#80111,#80112,#80113,#80114,#80115,#80116,#80117,#80118,#80119,
#80120,#80121,#80122,#80123,#80124,#80125,#80126,#80127,#80128,#80129,#80130,
#80131,#80132,#80133,#80134,#80135,#80136,#80137,#80138,#80139,#80140,#80141,
#80142,#80143,#80144,#80145,#80146,#80147,#80148,#80149,#80150,#80151,#80152,
#80153,#80154,#80155,#80156,#80157,#80158,#80159,#80160,#80161,#80162,#80163,
#80164,#80165,#80166,#80167,#80168,#80169,#80170,#80171,#80172,#80173,#80174,
#80175,#80176,#80177,#80178,#80179,#80180,#80181,#80182,#80183,#80184,#80185,
#80186,#80187,#80188,#80189,#80190,#80191,#80192,#80193,#80194,#80195,#80196,
#80197,#80198,#80199,#80200,#80201,#80202,#80203,#80204,#80205,#80206,#80207,
#80208,#80209,#80210,#80211,#80212,#80213,#80214,#80215,#80216,#80217,#80218,
#80219,#80220,#80221,#80222,#80223,#80224,#80225,#80226,#80227,#80228,#80229,
#80230,#80231,#80232,#80233,#80234,#80235,#80236,#80237,#80238,#80239,#80240,
#80241,#80242,#80243,#80244,#80245,#80246,#80247,#80248,#80249,#80250,#80251,
#80252,#80253,#80254,#80255,#80256,#80257,#80258,#80259,#80260,#80261,#80262,
#80263,#80264,#80265,#80266,#80267,#80268,#80269,#80270,#80271,#80272,#80273,
#80274,#80275,#80276,#80277,#80278,#80279,#80280),.UNSPECIFIED.,.F.,.F.,
(4,2,2,2,2,2,2,2,2,2,2,2,2,2,2,2,2,2,2,2,2,2,2,2,2,2,2,2,2,2,2,2,2,2,2,
2,2,2,2,2,2,2,2,2,2,2,2,2,2,2,2,2,2,2,2,2,2,2,2,2,2,2,2,2,2,2,2,2,2,2,2,
2,2,2,2,2,2,2,2,2,2,2,2,2,2,2,2,2,2,2,2,2,2,2,2,2,2,2,2,2,2,2,2,2,2,2,2,
2,2,2,2,2,2,2,2,2,2,2,2,2,2,2,2,2,2,2,2,2,2,2,2,2,2,2,2,2,2,4),(-1.40850074877309,
-1.39306820108003,-1.3827203300755,-1.37946735532854,-1.37739307038897,
-1.37545272476306,-1.37291376930828,-1.36862650202268,-1.33404472929969,
-1.2780780617487,-1.27380416440126,-1.27213256037046,-1.27112051463128,
-1.27001816035819,-1.26845321514756,-1.26454062554833,-1.24532800378349,
-1.18895312087029,-1.17210784928932,-1.16849108707793,-1.16612695367344,
-1.16421312881994,-1.16202094134709,-1.15823458076248,-1.14198762558551,
-1.08451185183594,-1.07953977447776,-1.06355442055558,-1.06093604447996,
-1.05958897221224,-1.05851763000277,-1.05726060533859,-1.05498547659474,
-1.04363391000168,-1.01755068902743,-0.964680736697037,-0.957777654122178,
-0.954909579772716,-0.953116350836811,-0.951155071172475,-0.948448931051755,
-0.942030686282602,-0.91345622310966,-0.862261700840353,-0.851098435335316,
-0.848945111478426,-0.847586697714472,-0.846514564852924,-0.845266070101644,
-0.843030061950331,-0.83233735008917,-0.808752957034694,-0.75217190320003,
-0.74560833398379,-0.743078737091019,-0.741255317044758,-0.739315192052921,
-0.736732877379483,-0.731018769371518,-0.708011392560211,-0.67498765768642,
-0.653828795219877,-0.639433447422016,-0.637109964437036,-0.635715473518186,
-0.634637223207563,-0.633426814054773,-0.631363245007312,-0.623093503649382,
-0.607315068087108,-0.565213967485415,-0.537106673358644,-0.532956862476877,
-0.530458132935264,-0.528524275512585,-0.526432936315915,-0.523101960962362,
-0.512049399581106,-0.493811250405697,-0.444967537422689,-0.427675161974073,
-0.425006237327776,-0.42364841644425,-0.422576429706423,-0.42132773562145,
-0.419090452187719,-0.408374313349663,-0.384702628642232,-0.328266125886046,
-0.321688290186996,-0.319156563088247,-0.317332702453529,-0.315393120830567,
-0.312813260737509,-0.307111715066948,-0.284195963295902,-0.233340123968605,
-0.231253244450221,-0.215570925639742,-0.212986407779205,-0.211661411573052,
-0.210640645945836,-0.21063259767656,-0.210624720817426,-0.210617004697119,
-0.210609439587844,-0.210602016435957,-0.210594726820411,-0.210587562955973,
-0.210580517691847,-0.210573584297352,-0.210566756412456,-0.210560028131177,
-0.210553393949895,-0.210546848679633,-0.210540387430724,-0.210534005674419,
-0.210527698994381,-0.210521463257463,-0.210515294582247,-0.210509189323113,
-0.21050314392979,-0.210497155008098,-0.210491219479333,-0.210485334399849,
-0.210479496741158,-0.20921701718876,-0.206832550359035,-0.19334069960194,
-0.157525544287272,-0.113371397423326,-0.109091499988174,-0.106554894876312,
-0.104615171834106,-0.102540411049315,-0.0992842990850559,-0.0889060651941913,
-0.0749176319822858),.UNSPECIFIED.);
#833=B_SPLINE_CURVE_WITH_KNOTS('',3,(#80281,#80282,#80283,#80284,#80285,
#80286,#80287,#80288,#80289,#80290,#80291,#80292,#80293,#80294,#80295,#80296,
#80297,#80298,#80299,#80300,#80301,#80302,#80303,#80304,#80305,#80306,#80307,
#80308,#80309,#80310,#80311,#80312,#80313,#80314,#80315,#80316,#80317,#80318,
#80319,#80320,#80321,#80322,#80323,#80324,#80325,#80326,#80327,#80328,#80329,
#80330,#80331,#80332,#80333,#80334,#80335,#80336,#80337,#80338,#80339,#80340,
#80341,#80342,#80343,#80344,#80345,#80346,#80347,#80348,#80349,#80350,#80351,
#80352,#80353,#80354,#80355,#80356,#80357,#80358,#80359,#80360,#80361,#80362,
#80363,#80364,#80365,#80366,#80367,#80368,#80369,#80370,#80371,#80372,#80373,
#80374,#80375,#80376,#80377,#80378,#80379,#80380,#80381,#80382,#80383,#80384,
#80385,#80386,#80387,#80388,#80389,#80390,#80391,#80392,#80393,#80394,#80395,
#80396,#80397,#80398,#80399,#80400,#80401,#80402,#80403,#80404,#80405,#80406,
#80407,#80408,#80409,#80410,#80411,#80412,#80413,#80414,#80415,#80416,#80417,
#80418,#80419,#80420,#80421,#80422,#80423,#80424,#80425,#80426,#80427,#80428,
#80429,#80430,#80431,#80432,#80433,#80434,#80435,#80436,#80437,#80438,#80439,
#80440,#80441,#80442,#80443,#80444,#80445,#80446,#80447,#80448,#80449,#80450,
#80451,#80452,#80453,#80454,#80455,#80456,#80457,#80458,#80459,#80460,#80461,
#80462,#80463,#80464,#80465,#80466,#80467,#80468,#80469,#80470,#80471,#80472,
#80473,#80474,#80475,#80476,#80477,#80478,#80479,#80480,#80481,#80482,#80483,
#80484,#80485,#80486,#80487,#80488,#80489,#80490,#80491,#80492,#80493,#80494,
#80495,#80496,#80497,#80498,#80499,#80500,#80501,#80502,#80503,#80504,#80505,
#80506,#80507,#80508,#80509,#80510),.UNSPECIFIED.,.F.,.F.,(4,2,2,2,2,2,
2,2,2,2,2,2,2,2,2,2,2,2,2,2,2,2,2,2,2,2,2,2,2,2,2,2,2,2,2,2,2,2,2,2,2,2,
2,2,2,2,2,2,2,2,2,2,2,2,2,2,2,2,2,2,2,2,2,2,2,2,2,2,2,2,2,2,2,2,2,2,2,2,
2,2,2,2,2,2,2,2,2,2,2,2,2,2,2,2,2,2,2,2,2,2,2,2,2,2,2,2,2,2,2,2,2,2,2,2,
4),(-2.59360340364756,-2.57256138631712,-2.5511722392252,-2.52301550873145,
-2.51638365243548,-2.51424433113592,-2.51215404354415,-2.51021879696438,
-2.5077149507316,-2.50354943372637,-2.47488951927506,-2.44415061377801,
-2.42040053984527,-2.40967571461453,-2.40744772913276,-2.40619083706372,
-2.40511921430145,-2.40377128206805,-2.40114974517762,-2.38511582430331,
-2.37974749555331,-2.33011817380235,-2.3073303447698,-2.30312526162724,
-2.30079622950563,-2.29888405526289,-2.29666371272857,-2.29285290562998,
-2.27799414844433,-2.26577003553844,-2.2101296064671,-2.19775202491306,
-2.19542091390671,-2.1941515954388,-2.19308083930896,-2.19174840654282,
-2.18968045830186,-2.17983290835504,-2.12787407010181,-2.0986295662347,
-2.09213164788723,-2.08941174157444,-2.08744763161007,-2.08565671622647,
-2.08280295027271,-2.07598897796227,-2.02201046904536,-1.99670885595042,
-1.98555634046624,-1.98329240682838,-1.98203764946754,-1.98096585615763,
-1.97961516960757,-1.97698077634107,-1.96061862186094,-1.95275972718494,
-1.9113643904438,-1.89271030025426,-1.8814787043257,-1.87812784636064,-1.87603163679148,
-1.87409844819305,-1.87160781687123,-1.8674871386554,-1.84053896816075,
-1.79860981765746,-1.78184881779291,-1.77323763734782,-1.77114615782812,
-1.76992929814559,-1.768852010821,-1.76746740761802,-1.76517834314845,-1.75150239063663,
-1.74978272647663,-1.70241634583266,-1.67144183938627,-1.66698984977577,
-1.6646542310998,-1.66274174095907,-1.66052676672508,-1.65673920557658,
-1.64214457813894,-1.62987905485822,-1.58946800527114,-1.57061431348597,
-1.56131551653981,-1.55917223486231,-1.55794395335048,-1.55686886081234,
-1.55547996957127,-1.55256526197488,-1.52372679175007,-1.48561706592977,
-1.4680913190089,-1.45735013842797,-1.45405245658675,-1.45196804348015,
-1.45003096048238,-1.44751443176755,-1.44330518777702,-1.41283118821453,
-1.36760503613842,-1.35571247943924,-1.35117739054435,-1.34786898136193,
-1.34640649833679,-1.34532179526139,-1.3441329069539,-1.34216696055788,
-1.33576185377284,-1.33420594521446,-1.31961940691524,-1.26057787761394,
-1.25976235679197),.UNSPECIFIED.);
#834=B_SPLINE_CURVE_WITH_KNOTS('',3,(#80516,#80517,#80518,#80519,#80520,
#80521,#80522,#80523),.UNSPECIFIED.,.F.,.F.,(4,2,2,4),(-0.0748537112472781,
-0.0742481380771646,-0.0252918457270349,-0.000629465073284334),
 .UNSPECIFIED.);
#835=B_SPLINE_CURVE_WITH_KNOTS('',3,(#80524,#80525,#80526,#80527,#80528,
#80529,#80530,#80531,#80532,#80533,#80534,#80535,#80536,#80537,#80538,#80539,
#80540,#80541,#80542,#80543,#80544,#80545,#80546,#80547,#80548,#80549,#80550,
#80551,#80552,#80553,#80554,#80555,#80556,#80557,#80558,#80559,#80560,#80561,
#80562,#80563,#80564,#80565,#80566,#80567,#80568,#80569,#80570,#80571,#80572,
#80573,#80574,#80575,#80576,#80577,#80578,#80579,#80580,#80581,#80582,#80583,
#80584,#80585,#80586,#80587,#80588,#80589,#80590,#80591,#80592,#80593,#80594,
#80595,#80596,#80597,#80598,#80599,#80600,#80601,#80602,#80603,#80604,#80605,
#80606,#80607,#80608,#80609,#80610,#80611,#80612,#80613,#80614,#80615,#80616,
#80617,#80618,#80619,#80620,#80621,#80622,#80623,#80624,#80625,#80626,#80627,
#80628,#80629,#80630,#80631,#80632,#80633,#80634,#80635,#80636,#80637,#80638,
#80639,#80640,#80641,#80642,#80643,#80644,#80645,#80646,#80647,#80648,#80649,
#80650,#80651,#80652,#80653,#80654,#80655,#80656,#80657,#80658,#80659,#80660,
#80661,#80662,#80663,#80664,#80665,#80666,#80667,#80668,#80669,#80670,#80671,
#80672,#80673,#80674,#80675,#80676,#80677,#80678,#80679,#80680,#80681,#80682,
#80683,#80684,#80685,#80686,#80687,#80688,#80689,#80690,#80691,#80692,#80693,
#80694,#80695,#80696,#80697,#80698,#80699,#80700,#80701,#80702,#80703,#80704,
#80705,#80706,#80707,#80708,#80709,#80710,#80711,#80712,#80713,#80714,#80715,
#80716,#80717,#80718,#80719,#80720,#80721,#80722,#80723,#80724,#80725,#80726,
#80727,#80728,#80729,#80730,#80731,#80732,#80733,#80734,#80735,#80736,#80737,
#80738,#80739,#80740,#80741,#80742,#80743,#80744,#80745,#80746,#80747,#80748,
#80749,#80750,#80751,#80752,#80753,#80754,#80755,#80756,#80757,#80758,#80759,
#80760,#80761,#80762,#80763,#80764,#80765,#80766,#80767,#80768,#80769,#80770,
#80771,#80772,#80773,#80774,#80775,#80776,#80777,#80778,#80779,#80780,#80781),
 .UNSPECIFIED.,.F.,.F.,(4,2,2,2,2,2,2,2,2,2,2,2,2,2,2,2,2,2,2,2,2,2,2,2,
2,2,2,2,2,2,2,2,2,2,2,2,2,2,2,2,2,2,2,2,2,2,2,2,2,2,2,2,2,2,2,2,2,2,2,2,
2,2,2,2,2,2,2,2,2,2,2,2,2,2,2,2,2,2,2,2,2,2,2,2,2,2,2,2,2,2,2,2,2,2,2,2,
2,2,2,2,2,2,2,2,2,2,2,2,2,2,2,2,2,2,2,2,2,2,2,2,2,2,2,2,2,2,2,2,4),(-2.66787357995012,
-2.66007952305088,-2.6547829299014,-2.65233947880885,-2.65045756852206,
-2.64861680673795,-2.64679034936771,-2.64424988281189,-2.63905856459427,
-2.62654797522341,-2.57487722209167,-2.55603430300991,-2.54673913222438,
-2.54459620358012,-2.5433680465749,-2.54229301224663,-2.54090412918185,
-2.53798920207424,-2.50829197952501,-2.45784167081142,-2.44835244368186,
-2.44374506839699,-2.4399658886159,-2.43779513881799,-2.43777944411622,
-2.43776319681168,-2.43774637681734,-2.43772896331178,-2.43771093465628,
-2.43769226847276,-2.43767294154989,-2.43765292981784,-2.43763220836344,
-2.43761075138144,-2.43758853216956,-2.43756552233064,-2.43754548574042,
-2.43752213510058,-2.43749492833802,-2.43746323740148,-2.43742633595271,
-2.43738338573796,-2.43732917339247,-2.43538841738136,-2.43284636145566,
-2.42854811310968,-2.3934263502408,-2.34446749666977,-2.33476696161901,
-2.33259567850242,-2.33136141126727,-2.33028756323901,-2.32890877629817,
-2.3260448467984,-2.29008787484562,-2.2573219623038,-2.23476228845003,-2.22910880690954,
-2.22653758761028,-2.22459917777942,-2.22277251411468,-2.22023063764096,
-2.21358963927326,-2.15778389595365,-2.13372116995794,-2.12289772429747,
-2.12065375760462,-2.11940352527556,-2.11833157456533,-2.11697553259889,
-2.11482997417052,-2.10379328073334,-2.0525752023922,-2.02386569585539,
-2.0174319174313,-2.01472320811927,-2.0127615134479,-2.01096890432522,-2.00810398368554,
-2.00121966482396,-1.94814357879202,-1.92223606838301,-1.91092874707077,
-1.90865624862904,-1.90739982387573,-1.90632847849168,-1.9049807410111,
-1.90235912942254,-1.88631694266447,-1.8810260332003,-1.86644143482478,
-1.83354904035393,-1.81698193268487,-1.80666937147902,-1.80342036504989,
-1.80134689793032,-1.79940611478273,-1.79686485256737,-1.79256980511797,
-1.75745725127151,-1.70855188049012,-1.69878122353251,-1.69660497181993,
-1.69536953386231,-1.69429572638613,-1.69291837619435,-1.69006220057868,
-1.66726170284572,-1.61165236203527,-1.59564067734481,-1.59187115493372,
-1.58968264924329,-1.58776841522675,-1.58539909578318,-1.58176566734115,
-1.5646682505217,-1.55659954196284,-1.52178855986863,-1.49773837571906,
-1.48691856672895,-1.48467491309625,-1.48342479338141,-1.48235290111825,
-1.4809968841986,-1.47833656340552,-1.46128286132611,-1.44267045856224,
-1.40971371125424,-1.40850074877309),.UNSPECIFIED.);
#836=B_SPLINE_CURVE_WITH_KNOTS('',3,(#80783,#80784,#80785,#80786,#80787,
#80788,#80789,#80790,#80791,#80792,#80793,#80794,#80795,#80796,#80797,#80798,
#80799,#80800,#80801,#80802,#80803,#80804,#80805,#80806,#80807,#80808,#80809,
#80810,#80811,#80812,#80813,#80814,#80815,#80816,#80817,#80818,#80819,#80820,
#80821,#80822,#80823,#80824,#80825,#80826,#80827,#80828,#80829,#80830,#80831,
#80832,#80833,#80834,#80835,#80836,#80837,#80838,#80839,#80840,#80841,#80842,
#80843,#80844,#80845,#80846,#80847,#80848,#80849,#80850,#80851,#80852,#80853,
#80854,#80855,#80856,#80857,#80858,#80859,#80860,#80861,#80862,#80863,#80864,
#80865,#80866,#80867,#80868,#80869,#80870,#80871,#80872,#80873,#80874,#80875,
#80876,#80877,#80878,#80879,#80880,#80881,#80882,#80883,#80884,#80885,#80886,
#80887,#80888,#80889,#80890,#80891,#80892,#80893,#80894,#80895,#80896,#80897,
#80898,#80899,#80900,#80901,#80902,#80903,#80904,#80905,#80906,#80907,#80908,
#80909,#80910,#80911,#80912,#80913,#80914,#80915,#80916,#80917,#80918,#80919,
#80920,#80921,#80922,#80923,#80924,#80925,#80926,#80927,#80928,#80929,#80930,
#80931,#80932,#80933,#80934,#80935,#80936,#80937,#80938,#80939,#80940,#80941,
#80942,#80943,#80944,#80945,#80946,#80947,#80948,#80949,#80950,#80951,#80952,
#80953,#80954,#80955,#80956,#80957,#80958,#80959,#80960,#80961,#80962,#80963,
#80964,#80965,#80966,#80967,#80968,#80969,#80970,#80971,#80972,#80973,#80974,
#80975,#80976,#80977,#80978,#80979,#80980,#80981,#80982,#80983,#80984,#80985,
#80986,#80987,#80988,#80989,#80990,#80991,#80992),.UNSPECIFIED.,.F.,.F.,
(4,2,2,2,2,2,2,2,2,2,2,2,2,2,2,2,2,2,2,2,2,2,2,2,2,2,2,2,2,2,2,2,2,2,2,
2,2,2,2,2,2,2,2,2,2,2,2,2,2,2,2,2,2,2,2,2,2,2,2,2,2,2,2,2,2,2,2,2,2,2,2,
2,2,2,2,2,2,2,2,2,2,2,2,2,2,2,2,2,2,2,2,2,2,2,2,2,2,2,2,2,2,2,2,2,4),(-1.25976235679197,
-1.24626820017445,-1.24250651621246,-1.24029768477833,-1.23838503090232,
-1.236042305457,-1.23155538041799,-1.19919364072031,-1.15901211212556,-1.15407926751949,
-1.13812902112765,-1.13551244877831,-1.13416572897147,-1.13309436405029,
-1.13183696125577,-1.12956025357522,-1.11818237288597,-1.09199616666393,
-1.03926923928351,-1.0323550250493,-1.02948503966214,-1.02769140453988,
-1.02573031367983,-1.02302559328425,-1.01661619053952,-0.988116890300663,
-0.937184400075926,-0.925703478976986,-0.923531070722116,-0.922166818820405,
-0.921094174941895,-0.919849766402907,-0.917632613690453,-0.907242331803809,
-0.88474480639707,-0.826437139346686,-0.820077536526286,-0.817581369715969,
-0.815766632341883,-0.813821312867422,-0.811207056028172,-0.805316664753698,
-0.780975561266437,-0.730307518474436,-0.714076158412379,-0.711447501238598,
-0.710098232471539,-0.709026765673658,-0.707771472672896,-0.705504239768999,
-0.694289042834435,-0.668738500796957,-0.615102074242418,-0.608259444881277,
-0.605401353355504,-0.603609960979995,-0.601647139746122,-0.598932347283126,
-0.592462547390376,-0.538190467564313,-0.502341470790713,-0.49948276983982,
-0.498104964751824,-0.497031157507482,-0.495796128800669,-0.493621562090834,
-0.483874740392211,-0.434926281688211,-0.399782672617695,-0.395494935780452,
-0.392955909870843,-0.391015619219038,-0.3889414977907,-0.385688997314133,
-0.375344394068019,-0.358708143016554,-0.325787971312303,-0.307705323540847,
-0.290152337107941,-0.28747409124646,-0.286114285592324,-0.285042149979008,
-0.283794908271799,-0.281564257964448,-0.270955442677452,-0.247674379497308,
-0.191965057539896,-0.184499505664943,-0.181536909186454,-0.179726412110841,
-0.177896471607758,-0.175389977398866,-0.170058138140225,-0.16297530619806,
-0.145592391782818,-0.0967472308571914,-0.0782163418531925,-0.0754719491544447,
-0.0741169405276754,-0.0730452173091221,-0.0717945786023242,-0.0695481925536985,
-0.0586810442108745,-0.0344507151062333,-0.000629544781513296),
 .UNSPECIFIED.);
#837=B_SPLINE_CURVE_WITH_KNOTS('',3,(#80993,#80994,#80995,#80996,#80997,
#80998,#80999,#81000,#81001,#81002,#81003,#81004,#81005,#81006,#81007,#81008,
#81009,#81010,#81011,#81012,#81013,#81014),.UNSPECIFIED.,.F.,.F.,(4,2,2,
2,2,2,2,2,2,2,4),(-2.6677880043013,-2.64246090365341,-2.63933381754846,
-2.63718766808863,-2.63538680183029,-2.63347278998466,-2.63110354900661,
-2.62746987279902,-2.6103639371884,-2.59817297007628,-2.59336440692509),
 .UNSPECIFIED.);
#838=B_SPLINE_CURVE_WITH_KNOTS('',3,(#81019,#81020,#81021,#81022,#81023,
#81024,#81025,#81026,#81027,#81028,#81029,#81030,#81031,#81032,#81033,#81034,
#81035,#81036,#81037,#81038,#81039,#81040,#81041,#81042,#81043,#81044,#81045,
#81046,#81047,#81048,#81049,#81050,#81051,#81052,#81053,#81054,#81055,#81056,
#81057,#81058,#81059,#81060,#81061,#81062,#81063,#81064,#81065,#81066,#81067,
#81068,#81069,#81070,#81071,#81072,#81073,#81074,#81075,#81076,#81077,#81078,
#81079,#81080,#81081,#81082,#81083,#81084,#81085,#81086,#81087,#81088,#81089,
#81090,#81091,#81092,#81093,#81094,#81095,#81096,#81097,#81098,#81099,#81100,
#81101,#81102,#81103,#81104,#81105,#81106,#81107,#81108,#81109,#81110,#81111,
#81112,#81113,#81114,#81115,#81116,#81117,#81118,#81119,#81120,#81121,#81122,
#81123,#81124,#81125,#81126,#81127,#81128,#81129,#81130,#81131,#81132,#81133,
#81134,#81135,#81136,#81137,#81138,#81139,#81140,#81141,#81142,#81143,#81144,
#81145,#81146,#81147,#81148,#81149,#81150,#81151,#81152,#81153,#81154,#81155,
#81156,#81157,#81158,#81159,#81160,#81161,#81162,#81163,#81164,#81165,#81166,
#81167,#81168,#81169,#81170,#81171,#81172,#81173,#81174,#81175,#81176,#81177,
#81178,#81179,#81180,#81181,#81182,#81183,#81184,#81185,#81186,#81187,#81188,
#81189,#81190,#81191,#81192,#81193,#81194,#81195,#81196,#81197,#81198,#81199,
#81200,#81201,#81202,#81203,#81204,#81205,#81206,#81207,#81208,#81209,#81210,
#81211,#81212,#81213,#81214,#81215,#81216,#81217,#81218,#81219,#81220,#81221,
#81222,#81223,#81224,#81225,#81226,#81227,#81228,#81229,#81230,#81231,#81232,
#81233,#81234,#81235,#81236,#81237,#81238,#81239,#81240,#81241,#81242,#81243,
#81244,#81245,#81246,#81247,#81248,#81249,#81250,#81251,#81252),
 .UNSPECIFIED.,.F.,.F.,(4,2,2,2,2,2,2,2,2,2,2,2,2,2,2,2,2,2,2,2,2,2,2,2,
2,2,2,2,2,2,2,2,2,2,2,2,2,2,2,2,2,2,2,2,2,2,2,2,2,2,2,2,2,2,2,2,2,2,2,2,
2,2,2,2,2,2,2,2,2,2,2,2,2,2,2,2,2,2,2,2,2,2,2,2,2,2,2,2,2,2,2,2,2,2,2,2,
2,2,2,2,2,2,2,2,2,2,2,2,2,2,2,2,2,2,2,2,4),(-1.40847046428017,-1.40132352298175,
-1.37516890792839,-1.36379827702942,-1.36152197446538,-1.36026464062407,
-1.35919324415307,-1.35784636364615,-1.35522912551683,-1.33926697255163,
-1.33432292216282,-1.32867694362814,-1.28171652932453,-1.28027334419647,
-1.26123206893809,-1.25747072348756,-1.25506190165986,-1.25314412556238,
-1.25098193577219,-1.24733221406709,-1.23288124413848,-1.18249242530521,
-1.15282398962037,-1.14990947138451,-1.14852069375532,-1.14744569607883,
-1.14621753994888,-1.1440745024417,-1.13477745886532,-1.11592580700965,
-1.07547219843435,-1.06319339613209,-1.04861347491532,-1.04482746730749,
-1.04261299377957,-1.04070068826315,-1.03836498344053,-1.03391186611421,
-1.00287554051865,-0.954897464000928,-0.940308394020928,-0.937976019532825,
-0.936578771059989,-0.93549996646566,-0.934290695070962,-0.93223296160082,
-0.924037446645905,-0.908471043793413,-0.86688692951543,-0.837982836940759,
-0.833811356119599,-0.831306001341352,-0.829370801191866,-0.827281764944157,
-0.823962531284684,-0.813022789874797,-0.795045951150402,-0.744623147091577,
-0.728417163136248,-0.725789283072615,-0.72444008630442,-0.723368505314425,
-0.722112880174972,-0.71984454505754,-0.708613735516601,-0.683004782707691,
-0.629442188046572,-0.6225921673684,-0.619732647821296,-0.617940842434842,
-0.615977957395679,-0.613263791885522,-0.606798897371197,-0.552722670112585,
-0.516660413468051,-0.51380066915979,-0.512422560592397,-0.511348610414594,
-0.510113522915429,-0.507939104981787,-0.498197107877221,-0.449237654418865,
-0.414102807337012,-0.40980635345955,-0.40726464369366,-0.405323729275715,
-0.403250325111179,-0.400001840352817,-0.389694415829426,-0.373141176416832,
-0.340287500554374,-0.32728540853776,-0.304664045697818,-0.301812381731855,
-0.300435946598413,-0.299362255983898,-0.298126286934198,-0.295947492322959,
-0.286139094692546,-0.237241731478906,-0.202131567716715,-0.197834504820012,
-0.195292756248984,-0.193351997280235,-0.191344263213684,-0.188242470263319,
-0.18461585140243,-0.177819650839178,-0.161438226066528,-0.128729471565566,
-0.092700370640288,-0.0898402863548513,-0.088462274498264,-0.0873885219422777,
-0.0861537996592544,-0.0839803541722877,-0.0748537112472781),
 .UNSPECIFIED.);
#839=B_SPLINE_CURVE_WITH_KNOTS('',3,(#81253,#81254,#81255,#81256,#81257,
#81258,#81259,#81260,#81261,#81262,#81263,#81264,#81265,#81266,#81267,#81268,
#81269,#81270,#81271,#81272,#81273,#81274,#81275,#81276,#81277,#81278,#81279,
#81280,#81281,#81282,#81283,#81284,#81285,#81286,#81287,#81288,#81289,#81290,
#81291,#81292,#81293,#81294,#81295,#81296,#81297,#81298,#81299,#81300,#81301,
#81302,#81303,#81304,#81305,#81306,#81307,#81308,#81309,#81310,#81311,#81312,
#81313,#81314,#81315,#81316,#81317,#81318,#81319,#81320,#81321,#81322,#81323,
#81324,#81325,#81326,#81327,#81328,#81329,#81330,#81331,#81332,#81333,#81334,
#81335,#81336,#81337,#81338,#81339,#81340,#81341,#81342,#81343,#81344,#81345,
#81346,#81347,#81348,#81349,#81350,#81351,#81352,#81353,#81354,#81355,#81356,
#81357,#81358,#81359,#81360,#81361,#81362,#81363,#81364,#81365,#81366,#81367,
#81368,#81369,#81370,#81371,#81372,#81373,#81374,#81375,#81376,#81377,#81378,
#81379,#81380,#81381,#81382,#81383,#81384,#81385,#81386,#81387,#81388,#81389,
#81390,#81391,#81392,#81393,#81394,#81395,#81396,#81397,#81398,#81399,#81400,
#81401,#81402,#81403,#81404,#81405,#81406,#81407,#81408,#81409,#81410,#81411,
#81412,#81413,#81414,#81415,#81416,#81417,#81418,#81419,#81420,#81421,#81422,
#81423,#81424,#81425,#81426,#81427,#81428,#81429,#81430,#81431,#81432,#81433,
#81434,#81435,#81436,#81437,#81438,#81439,#81440,#81441,#81442,#81443,#81444,
#81445,#81446,#81447,#81448,#81449,#81450,#81451,#81452,#81453,#81454,#81455,
#81456,#81457,#81458,#81459,#81460,#81461,#81462,#81463,#81464,#81465,#81466,
#81467,#81468,#81469,#81470,#81471,#81472,#81473,#81474,#81475,#81476,#81477,
#81478,#81479,#81480,#81481,#81482,#81483,#81484,#81485,#81486,#81487,#81488,
#81489,#81490,#81491,#81492,#81493,#81494,#81495,#81496,#81497,#81498,#81499,
#81500,#81501,#81502,#81503,#81504,#81505,#81506,#81507,#81508,#81509,#81510,
#81511,#81512,#81513,#81514,#81515,#81516,#81517,#81518,#81519,#81520,#81521,
#81522,#81523,#81524),.UNSPECIFIED.,.F.,.F.,(4,2,2,2,2,2,2,2,2,2,2,2,2,
2,2,2,2,2,2,2,2,2,2,2,2,2,2,2,2,2,2,2,2,2,2,2,2,2,2,2,2,2,2,2,2,2,2,2,2,
2,2,2,2,2,2,2,2,2,2,2,2,2,2,2,2,2,2,2,2,2,2,2,2,2,2,2,2,2,2,2,2,2,2,2,2,
2,2,2,2,2,2,2,2,2,2,2,2,2,2,2,2,2,2,2,2,2,2,2,2,2,2,2,2,2,2,2,2,2,2,2,2,
2,2,2,2,2,2,2,2,2,2,2,2,2,2,4),(-2.59336440692509,-2.55352828350367,-2.53505701142379,
-2.53122442869316,-2.52967258864427,-2.52857286897742,-2.52755811021205,
-2.52587166995057,-2.52150532217003,-2.47379324060003,-2.44450201015887,
-2.43448885743048,-2.42970049862564,-2.42580682697683,-2.42360320076253,
-2.42359053035804,-2.42357742258592,-2.4235638611813,-2.4235498292744,-2.42353530638362,
-2.42352027587282,-2.42350472032353,-2.42348861994496,-2.42347195416413,
-2.42345470152217,-2.42343683970557,-2.42341834549094,-2.42339919465093,
-2.42337936200965,-2.42335882136724,-2.42333754541899,-2.4233155057623,
-2.42329267219068,-2.4232733641008,-2.42325080766968,-2.42322445319372,
-2.42319365740929,-2.42315766767554,-2.42311560362571,-2.42306770789945,
-2.42112699268115,-2.41858504650969,-2.41428711006614,-2.37917263951499,
-2.33023652674197,-2.32051020260422,-2.31833716733843,-2.31710252607242,
-2.31602875148292,-2.31465058069139,-2.31178973116941,-2.27575005051651,
-2.22155102093976,-2.21514494306319,-2.2124410403361,-2.21048033165337,
-2.20868690476235,-2.20581693278741,-2.19890107411085,-2.14626117479252,
-2.1200537036965,-2.10867059178548,-2.10639388181172,-2.10513660242519,
-2.10406542169799,-2.10271902780342,-2.1001033673971,-2.08416512341129,
-2.07847906392991,-2.06417027831973,-2.03128355126708,-2.0147214613364,
-2.0044113905213,-2.00116283204631,-1.99908956992277,-1.99714892184211,
-1.99460775452005,-1.99031268376186,-1.95517547731458,-1.90618873829942,
-1.89651929532217,-1.89435012157751,-1.89311629951435,-1.89204235453933,
-1.89066280893114,-1.88843968609813,-1.87605207030594,-1.8729889090395,
-1.87279059541371,-1.86592304485023,-1.85219045972894,-1.8193075068519,
-1.80275161124286,-1.79244413964882,-1.78919573134311,-1.78712240432094,
-1.78518158257353,-1.78264002490765,-1.77834392916455,-1.74314884891007,
-1.69397734468337,-1.68451769984892,-1.68236311321726,-1.68113244848262,
-1.68005792827272,-1.67867327477203,-1.67577973947107,-1.6497449430723,
-1.61157746531009,-1.58254918462702,-1.57815351942445,-1.57582991862997,
-1.57391828909574,-1.57169413805559,-1.56786583439451,-1.5528043005564,
-1.50063521466255,-1.48178940586435,-1.47249345335754,-1.47035052877893,
-1.4691224038069,-1.4680474168998,-1.46665862069468,-1.46374396626898,-1.43369740855554,
-1.38235508191602,-1.36901471600201,-1.36545962391766,-1.36331844013418,
-1.36139713145788,-1.35895376713785,-1.35507915828794,-1.33400470217004,
-1.27618798964858,-1.26122697294337,-1.25979252647547),.UNSPECIFIED.);
#840=B_SPLINE_CURVE_WITH_KNOTS('',3,(#81530,#81531,#81532,#81533),
 .UNSPECIFIED.,.F.,.F.,(4,4),(120.339865595025,120.689851222995),
 .UNSPECIFIED.);
#841=B_SPLINE_CURVE_WITH_KNOTS('',3,(#81534,#81535,#81536,#81537,#81538,
#81539,#81540,#81541,#81542,#81543,#81544,#81545,#81546,#81547,#81548,#81549,
#81550,#81551,#81552,#81553,#81554,#81555,#81556,#81557,#81558,#81559,#81560,
#81561,#81562,#81563,#81564,#81565,#81566,#81567,#81568,#81569,#81570,#81571,
#81572,#81573,#81574,#81575,#81576,#81577,#81578,#81579,#81580,#81581,#81582,
#81583,#81584,#81585,#81586,#81587,#81588,#81589,#81590,#81591,#81592,#81593,
#81594,#81595,#81596,#81597,#81598,#81599,#81600,#81601,#81602,#81603,#81604,
#81605,#81606,#81607,#81608,#81609,#81610,#81611,#81612,#81613,#81614,#81615,
#81616,#81617,#81618,#81619,#81620,#81621,#81622,#81623,#81624,#81625,#81626,
#81627,#81628,#81629,#81630,#81631,#81632,#81633,#81634,#81635,#81636,#81637,
#81638,#81639,#81640,#81641,#81642,#81643,#81644,#81645,#81646,#81647,#81648,
#81649,#81650,#81651,#81652,#81653,#81654,#81655,#81656,#81657,#81658,#81659,
#81660,#81661,#81662,#81663,#81664,#81665,#81666,#81667,#81668,#81669,#81670,
#81671,#81672,#81673,#81674,#81675,#81676,#81677,#81678,#81679,#81680,#81681,
#81682,#81683,#81684,#81685,#81686,#81687,#81688,#81689,#81690,#81691,#81692,
#81693,#81694,#81695,#81696,#81697,#81698,#81699,#81700,#81701,#81702,#81703,
#81704,#81705,#81706,#81707,#81708,#81709,#81710,#81711,#81712,#81713,#81714,
#81715,#81716,#81717,#81718,#81719,#81720,#81721,#81722,#81723,#81724,#81725,
#81726,#81727,#81728,#81729,#81730,#81731,#81732,#81733,#81734,#81735,#81736,
#81737,#81738,#81739,#81740,#81741,#81742,#81743,#81744,#81745,#81746,#81747,
#81748,#81749,#81750,#81751),.UNSPECIFIED.,.F.,.F.,(4,2,2,2,2,2,2,2,2,2,
2,2,2,2,2,2,2,2,2,2,2,2,2,2,2,2,2,2,2,2,2,2,2,2,2,2,2,2,2,2,2,2,2,2,2,2,
2,2,2,2,2,2,2,2,2,2,2,2,2,2,2,2,2,2,2,2,2,2,2,2,2,2,2,2,2,2,2,2,2,2,2,2,
2,2,2,2,2,2,2,2,2,2,2,2,2,2,2,2,2,2,2,2,2,2,2,2,2,2,4),(-2.66761347800519,
-2.6433834721182,-2.63625151418383,-2.6344605986207,-2.63324562918053,-2.63223654706512,
-2.63116196370503,-2.62977592206083,-2.62687490453753,-2.59995438394439,
-2.58627120477344,-2.57475044801003,-2.54617410255535,-2.53227597603649,
-2.5286724497231,-2.52652058051867,-2.52460130391527,-2.52217626522362,
-2.5174445027455,-2.48000718468932,-2.42965580471258,-2.42318147430023,
-2.42128999998669,-2.42027902641582,-2.41920575391483,-2.41783408622734,
-2.41563718858464,-2.40380140420529,-2.34640651839376,-2.32984068112255,
-2.31952892163212,-2.31628017359891,-2.31420687278027,-2.31226624627227,
-2.30972519057587,-2.3054304953408,-2.2703212410984,-2.2214212514753,-2.21164967386911,
-2.20947348073862,-2.20823811664349,-2.20716439935445,-2.20578719881336,
-2.20293145037008,-2.1667815175419,-2.1340772828521,-2.11161423548992,-2.105973787024,
-2.10340493239071,-2.10146685306004,-2.09963943268177,-2.09709478730645,
-2.09043627800359,-2.03479837324969,-2.01062429006053,-1.99977076078248,
-1.99752493983372,-1.99627428726215,-1.99520235380513,-1.99384681784614,
-1.9911890366621,-1.97420781840533,-1.92397680279609,-1.90639062592672,
-1.89562347727925,-1.89232338664344,-1.8902387379499,-1.88830232422253,
-1.88578792521051,-1.88158501522212,-1.85135605137762,-1.79985750068206,
-1.78786948078818,-1.78555919209865,-1.78429455517402,-1.78322379469047,
-1.78188637381476,-1.77980165691238,-1.7697077673214,-1.76421756231126,
-1.75679091328359,-1.7432832209496,-1.71040118646671,-1.69384734487439,
-1.68354068589893,-1.6802922854624,-1.67821890379077,-1.67627798896135,
-1.67373624889946,-1.66943970920898,-1.63422230751653,-1.5849768578298,
-1.57559915897596,-1.57345035128136,-1.57222092901265,-1.57114615644823,
-1.56975941623923,-1.56751267435131,-1.55467956045432,-1.55251360859266,
-1.50523272964611,-1.47670829575112,-1.47029626611204,-1.46759105332923,
-1.46562983216923,-1.46383623793925,-1.4609666551701,-1.45405513324635,
-1.40847046428017),.UNSPECIFIED.);
#842=B_SPLINE_CURVE_WITH_KNOTS('',3,(#81753,#81754,#81755,#81756,#81757,
#81758,#81759,#81760,#81761,#81762,#81763,#81764,#81765,#81766,#81767,#81768,
#81769,#81770,#81771,#81772,#81773,#81774,#81775,#81776,#81777,#81778,#81779,
#81780,#81781,#81782,#81783,#81784,#81785,#81786,#81787,#81788,#81789,#81790,
#81791,#81792,#81793,#81794,#81795,#81796,#81797,#81798,#81799,#81800,#81801,
#81802,#81803,#81804,#81805,#81806,#81807,#81808,#81809,#81810,#81811,#81812,
#81813,#81814,#81815,#81816,#81817,#81818,#81819,#81820,#81821,#81822,#81823,
#81824,#81825,#81826,#81827,#81828,#81829,#81830,#81831,#81832,#81833,#81834,
#81835,#81836,#81837,#81838,#81839,#81840,#81841,#81842,#81843,#81844,#81845,
#81846,#81847,#81848,#81849,#81850,#81851,#81852,#81853,#81854,#81855,#81856,
#81857,#81858,#81859,#81860,#81861,#81862,#81863,#81864,#81865,#81866,#81867,
#81868,#81869,#81870,#81871,#81872,#81873,#81874,#81875,#81876,#81877,#81878,
#81879,#81880,#81881,#81882,#81883,#81884,#81885,#81886,#81887,#81888,#81889,
#81890,#81891,#81892,#81893,#81894,#81895,#81896,#81897,#81898,#81899,#81900,
#81901,#81902,#81903,#81904,#81905,#81906,#81907,#81908,#81909,#81910,#81911,
#81912,#81913,#81914,#81915,#81916,#81917,#81918,#81919,#81920,#81921,#81922,
#81923,#81924,#81925,#81926,#81927,#81928,#81929,#81930,#81931,#81932,#81933,
#81934,#81935,#81936,#81937,#81938,#81939,#81940,#81941,#81942,#81943,#81944,
#81945,#81946,#81947,#81948,#81949,#81950,#81951,#81952,#81953,#81954,#81955,
#81956,#81957,#81958,#81959,#81960,#81961,#81962,#81963,#81964,#81965,#81966,
#81967,#81968,#81969,#81970,#81971,#81972,#81973,#81974),.UNSPECIFIED.,
 .F.,.F.,(4,2,2,2,2,2,2,2,2,2,2,2,2,2,2,2,2,2,2,2,2,2,2,2,2,2,2,2,2,2,2,
2,2,2,2,2,2,2,2,2,2,2,2,2,2,2,2,2,2,2,2,2,2,2,2,2,2,2,2,2,2,2,2,2,2,2,2,
2,2,2,2,2,2,2,2,2,2,2,2,2,2,2,2,2,2,2,2,2,2,2,2,2,2,2,2,2,2,2,2,2,2,2,2,
2,2,2,2,2,2,2,4),(-1.25979252647547,-1.25887889341592,-1.25747705737434,
-1.25639764392859,-1.25519095057337,-1.25314477252933,-1.24508712466656,
-1.22990744614211,-1.19000994758103,-1.15896508172533,-1.15474340551486,
-1.15222338942829,-1.15028591448972,-1.14820333179291,-1.14491332875123,
-1.13423934940233,-1.11686744616279,-1.06816234198595,-1.06164762621188,
-1.04902404099949,-1.04678821408002,-1.04540474022874,-1.04433028019705,
-1.04309873277261,-1.04094033831612,-1.03142837623245,-0.982273139227336,
-0.947076376235956,-0.942779910067417,-0.940238221103645,-0.938297338737498,
-0.936223984487176,-0.932975610658268,-0.922668813952225,-0.906116845268339,
-0.873264580199634,-0.860348600354246,-0.837642694366873,-0.834789000078278,
-0.833412181479801,-0.832338472363633,-0.83110279901225,-0.828925284820705,
-0.819135261721587,-0.77022351376216,-0.735105339481279,-0.730810309447051,
-0.72826917455433,-0.726328545106829,-0.724255296039391,-0.7210067425078,
-0.710696472033711,-0.694136163459701,-0.661279012089867,-0.647506749294093,
-0.640733385971472,-0.638821061207603,-0.625183769865074,-0.62289719329886,
-0.621513569018754,-0.620436718197538,-0.619219996360079,-0.617127934419265,
-0.608503208895952,-0.591697035856527,-0.549706679495292,-0.52286696538262,
-0.518749929312503,-0.516260844577871,-0.514328456616962,-0.512232714107069,
-0.50888172952339,-0.497641368345566,-0.478966723314332,-0.438839923941719,
-0.41380087582269,-0.410918952487877,-0.409536720207729,-0.408462617229743,
-0.407230796527176,-0.405070307433445,-0.395523297753743,-0.346412592340616,
-0.311234327402151,-0.306939055184372,-0.304398034491327,-0.302457640524534,
-0.300384786772966,-0.297137152755538,-0.28683232985951,-0.270283175851369,
-0.237936898606343,-0.201815507226788,-0.198960473064593,-0.197583584042405,
-0.196557069340875,-0.195363682822098,-0.193380726592143,-0.190940963612911,
-0.185982559260592,-0.17243164223367,-0.149608806289563,-0.103071661430291,
-0.0958752135165292,-0.0929587241486494,-0.091156918417348,-0.0892033949999929,
-0.0865388798007457,-0.0803614985460654,-0.0537590801016044,-0.000629603543800122),
 .UNSPECIFIED.);
#843=B_SPLINE_CURVE_WITH_KNOTS('',3,(#81975,#81976,#81977,#81978,#81979,
#81980,#81981,#81982,#81983,#81984,#81985,#81986,#81987,#81988,#81989,#81990,
#81991,#81992,#81993,#81994,#81995,#81996,#81997,#81998),.UNSPECIFIED.,
 .F.,.F.,(4,2,2,2,2,2,2,2,2,2,2,4),(-2.66790098184336,-2.65984464261496,
-2.65548769960189,-2.65407479042277,-2.65300760105439,-2.65197745200527,
-2.65079760878932,-2.64887250690142,-2.64280732657753,-2.64152539353864,
-2.63372545384238,-2.59364855829229),.UNSPECIFIED.);
#844=B_SPLINE_CURVE_WITH_KNOTS('',3,(#82004,#82005,#82006,#82007,#82008,
#82009,#82010,#82011,#82012,#82013,#82014,#82015,#82016),.UNSPECIFIED.,
 .F.,.F.,(4,3,3,3,4),(114.057240355702,114.163813747114,114.270250447716,
114.376547360525,114.406671945289),.UNSPECIFIED.);
#845=B_SPLINE_CURVE_WITH_KNOTS('',3,(#82017,#82018,#82019,#82020,#82021,
#82022,#82023,#82024,#82025,#82026),.UNSPECIFIED.,.F.,.F.,(4,1,1,1,1,1,
1,4),(114.406674973147,114.866191745616,115.865028195577,116.863864645539,
117.862701095501,118.861537545463,119.860373995425,120.339865595025),
 .UNSPECIFIED.);
#846=B_SPLINE_CURVE_WITH_KNOTS('',3,(#82027,#82028,#82029,#82030,#82031,
#82032,#82033,#82034,#82035,#82036,#82037,#82038,#82039,#82040,#82041,#82042,
#82043,#82044,#82045,#82046,#82047,#82048,#82049,#82050,#82051,#82052,#82053,
#82054,#82055,#82056,#82057,#82058,#82059,#82060,#82061,#82062,#82063,#82064,
#82065,#82066,#82067,#82068,#82069,#82070,#82071,#82072,#82073,#82074,#82075,
#82076,#82077,#82078,#82079,#82080,#82081,#82082,#82083,#82084,#82085,#82086,
#82087,#82088,#82089,#82090,#82091,#82092,#82093,#82094,#82095,#82096,#82097,
#82098,#82099,#82100,#82101,#82102,#82103,#82104,#82105,#82106,#82107,#82108,
#82109,#82110,#82111,#82112,#82113,#82114,#82115,#82116,#82117,#82118,#82119,
#82120,#82121,#82122,#82123,#82124,#82125,#82126,#82127,#82128,#82129,#82130,
#82131,#82132,#82133,#82134,#82135,#82136,#82137,#82138,#82139,#82140,#82141,
#82142,#82143,#82144,#82145,#82146,#82147,#82148,#82149,#82150,#82151,#82152,
#82153,#82154,#82155,#82156,#82157,#82158,#82159,#82160,#82161,#82162,#82163,
#82164,#82165,#82166,#82167,#82168,#82169,#82170,#82171,#82172,#82173,#82174,
#82175,#82176,#82177,#82178,#82179,#82180,#82181,#82182,#82183,#82184,#82185,
#82186,#82187,#82188,#82189,#82190,#82191,#82192,#82193,#82194,#82195,#82196,
#82197,#82198,#82199,#82200,#82201,#82202,#82203,#82204,#82205,#82206,#82207,
#82208,#82209,#82210,#82211,#82212,#82213,#82214,#82215,#82216,#82217,#82218,
#82219,#82220,#82221,#82222,#82223,#82224,#82225,#82226,#82227,#82228,#82229,
#82230,#82231,#82232,#82233,#82234,#82235,#82236,#82237,#82238,#82239,#82240,
#82241,#82242,#82243,#82244,#82245,#82246,#82247,#82248,#82249,#82250,#82251,
#82252,#82253,#82254,#82255,#82256,#82257,#82258,#82259,#82260,#82261,#82262,
#82263,#82264,#82265,#82266,#82267,#82268,#82269,#82270,#82271,#82272,#82273,
#82274,#82275,#82276,#82277,#82278,#82279,#82280,#82281,#82282,#82283,#82284,
#82285,#82286,#82287,#82288,#82289,#82290),.UNSPECIFIED.,.F.,.F.,(4,2,2,
2,2,2,2,2,2,2,2,2,2,2,2,2,2,2,2,2,2,2,2,2,2,2,2,2,2,2,2,2,2,2,2,2,2,2,2,
2,2,2,2,2,2,2,2,2,2,2,2,2,2,2,2,2,2,2,2,2,2,2,2,2,2,2,2,2,2,2,2,2,2,2,2,
2,2,2,2,2,2,2,2,2,2,2,2,2,2,2,2,2,2,2,2,2,2,2,2,2,2,2,2,2,2,2,2,2,2,2,2,
2,2,2,2,2,2,2,2,2,2,2,2,2,2,2,2,2,2,2,2,4),(-2.59364855829229,-2.5805250390893,
-2.56278409515015,-2.55194824308276,-2.54864010448277,-2.54655336619433,
-2.54461707343816,-2.54210575134297,-2.53791439225231,-2.50842858115089,
-2.46731095672715,-2.45187633184749,-2.44646213612818,-2.44386337344784,
-2.44175675651997,-2.44054411539259,-2.44054100113675,-2.44053786796906,
-2.44053471576331,-2.440531544221,-2.44052835331933,-2.44052514307576,-2.44052191317927,
-2.44051866364419,-2.44051539419197,-2.4405121047115,-2.44050879501797,
-2.44050546497834,-2.44050212737287,-2.44049877521803,-2.44049540179566,
-2.44049199573067,-2.43946512739101,-2.43808765114628,-2.43523064398115,
-2.39912900337228,-2.36640698650285,-2.3439172832933,-2.33827312953013,
-2.33570353886459,-2.33376529201392,-2.33193799891083,-2.32939398900985,
-2.32273989542432,-2.26705329049152,-2.2429091628729,-2.23206353727476,
-2.22981813779165,-2.22856755012391,-2.22749556769191,-2.22613983566474,
-2.22399542335479,-2.21297854205454,-2.16170673761884,-2.13301944249611,
-2.12658814075178,-2.12387975860036,-2.12191804118312,-2.12012523265721,
-2.11725960484551,-2.11037157391679,-2.0573357314304,-2.03139671812569,
-2.02008110211527,-2.01780803637586,-2.01655144579858,-2.01548004876671,
-2.01413236059077,-2.01151118107485,-1.99547737576824,-1.99012770017464,
-1.97558900395009,-1.94269530041915,-1.92612790666373,-1.91581505838574,
-1.9125659036276,-1.91049232794615,-1.90855143342184,-1.90601001128875,
-1.90171466200994,-1.86659546915743,-1.81767306039634,-1.80791878915001,
-1.80574357444182,-1.80450832216617,-1.80343441801579,-1.80205660640985,
-1.79919831262477,-1.76327229888415,-1.73048510814842,-1.70789681308268,
-1.70223904576694,-1.69966679498596,-1.69772798077336,-1.69590121023253,
-1.69335962498487,-1.68672200580071,-1.63085911057923,-1.59803594974168,
-1.5944896466977,-1.5929853778273,-1.59189393470636,-1.59086651402607,-1.58911619747208,
-1.58433683795399,-1.5471606601068,-1.49689563116333,-1.49049358079696,
-1.48778997636317,-1.48582897324537,-1.48403492493844,-1.48116319051874,
-1.47423911293729,-1.42167206835065,-1.39539895020632,-1.38399813355596,
-1.381720029709,-1.38046226719308,-1.37939084842721,-1.37804437606064,-1.37542921060009,
-1.35950919466378,-1.35500709880457,-1.33444481736832,-1.28609239079606,
-1.27894364697813,-1.2760345128509,-1.27423358169825,-1.27227811319839,
-1.26960574452449,-1.26338653378267,-1.25991862954624),.UNSPECIFIED.);
#847=B_SPLINE_CURVE_WITH_KNOTS('',3,(#82296,#82297,#82298,#82299,#82300,
#82301,#82302,#82303,#82304,#82305,#82306,#82307,#82308,#82309,#82310,#82311,
#82312,#82313,#82314,#82315),.UNSPECIFIED.,.F.,.F.,(4,2,2,2,2,2,2,2,2,4),
(-0.0747504805022791,-0.0610229393326167,-0.0562870043262844,-0.0545435809193945,
-0.0535177049891406,-0.0524257922462895,-0.0509174391141034,-0.0492296202934677,
-0.0462824094859165,-0.000629118857166747),.UNSPECIFIED.);
#848=B_SPLINE_CURVE_WITH_KNOTS('',3,(#82316,#82317,#82318,#82319,#82320,
#82321,#82322,#82323,#82324,#82325,#82326,#82327,#82328,#82329,#82330,#82331,
#82332,#82333,#82334,#82335,#82336,#82337,#82338,#82339,#82340,#82341,#82342,
#82343,#82344,#82345,#82346,#82347,#82348,#82349,#82350,#82351,#82352,#82353,
#82354,#82355,#82356,#82357,#82358,#82359,#82360,#82361,#82362,#82363,#82364,
#82365,#82366,#82367,#82368,#82369,#82370,#82371,#82372,#82373,#82374,#82375,
#82376,#82377,#82378,#82379,#82380,#82381,#82382,#82383,#82384,#82385,#82386,
#82387,#82388,#82389,#82390,#82391,#82392,#82393,#82394,#82395,#82396,#82397,
#82398,#82399,#82400,#82401,#82402,#82403,#82404,#82405,#82406,#82407,#82408,
#82409,#82410,#82411,#82412,#82413,#82414,#82415,#82416,#82417,#82418,#82419,
#82420,#82421,#82422,#82423,#82424,#82425,#82426,#82427,#82428,#82429,#82430,
#82431,#82432,#82433,#82434,#82435,#82436,#82437,#82438,#82439,#82440,#82441,
#82442,#82443,#82444,#82445,#82446,#82447,#82448,#82449,#82450,#82451,#82452,
#82453,#82454,#82455,#82456,#82457,#82458,#82459,#82460,#82461,#82462,#82463,
#82464,#82465,#82466,#82467,#82468,#82469,#82470,#82471,#82472,#82473,#82474,
#82475,#82476,#82477,#82478,#82479,#82480,#82481,#82482,#82483,#82484,#82485,
#82486,#82487,#82488,#82489,#82490,#82491,#82492,#82493,#82494,#82495,#82496),
 .UNSPECIFIED.,.F.,.F.,(4,3,3,3,3,3,3,3,3,3,3,3,3,3,3,3,3,3,3,3,3,3,3,3,
3,3,3,3,3,3,3,3,3,3,3,3,3,3,3,3,3,3,3,3,3,3,3,3,3,3,3,3,3,3,3,3,3,3,3,3,
4),(108.12348663811,108.225421296431,108.327291076164,108.429131491865,
108.530978014042,108.632930880402,108.734945943836,108.837130903885,108.873173045844,
108.976567782892,109.079809065007,109.1829290304,109.285983598609,109.389006806967,
109.492032649639,109.595165416418,109.698354507828,109.801726501209,109.872009495806,
109.975404232854,110.078645514969,110.181765480361,110.28482004857,110.387843256928,
110.490869099601,110.594001866379,110.697190957789,110.80056295117,110.870845945768,
110.974240682816,111.077481964931,111.180601930324,111.283656498532,111.38667970689,
111.489705549562,111.59283831634,111.69602740775,111.799399401132,111.86968239573,
111.973077132778,112.076318414893,112.179438380285,112.282492948494,112.385516156852,
112.488541999524,112.591674766302,112.694863857712,112.798235851094,112.868518845692,
112.97191358274,113.075154864855,113.178274830248,113.281329398457,113.384352606815,
113.487378449488,113.590511216266,113.693700307676,113.797072301057,113.867355295654,
113.974272639427,114.057240355702),.UNSPECIFIED.);
#849=B_SPLINE_CURVE_WITH_KNOTS('',3,(#82498,#82499,#82500,#82501,#82502,
#82503,#82504,#82505,#82506,#82507,#82508,#82509,#82510,#82511,#82512,#82513,
#82514,#82515,#82516,#82517,#82518,#82519,#82520,#82521,#82522,#82523,#82524,
#82525,#82526,#82527,#82528,#82529,#82530,#82531,#82532,#82533,#82534,#82535,
#82536,#82537,#82538,#82539,#82540,#82541,#82542,#82543,#82544,#82545,#82546,
#82547,#82548,#82549,#82550,#82551,#82552,#82553,#82554,#82555,#82556,#82557,
#82558,#82559,#82560,#82561,#82562,#82563,#82564,#82565,#82566,#82567,#82568,
#82569,#82570,#82571,#82572,#82573,#82574,#82575,#82576,#82577,#82578,#82579,
#82580,#82581,#82582,#82583,#82584,#82585,#82586,#82587,#82588,#82589,#82590,
#82591,#82592,#82593,#82594,#82595,#82596,#82597,#82598,#82599,#82600,#82601,
#82602,#82603,#82604,#82605,#82606,#82607,#82608,#82609,#82610,#82611,#82612,
#82613,#82614,#82615,#82616,#82617,#82618,#82619,#82620,#82621,#82622,#82623,
#82624,#82625,#82626,#82627,#82628,#82629,#82630,#82631,#82632,#82633,#82634,
#82635,#82636,#82637,#82638,#82639,#82640,#82641,#82642,#82643,#82644,#82645,
#82646,#82647,#82648,#82649,#82650,#82651,#82652,#82653,#82654,#82655,#82656,
#82657,#82658,#82659,#82660,#82661,#82662,#82663,#82664,#82665,#82666,#82667,
#82668,#82669,#82670,#82671,#82672,#82673,#82674,#82675,#82676,#82677,#82678,
#82679,#82680,#82681,#82682,#82683,#82684,#82685,#82686,#82687,#82688,#82689,
#82690,#82691,#82692,#82693,#82694,#82695,#82696,#82697,#82698,#82699,#82700,
#82701,#82702,#82703,#82704,#82705,#82706,#82707,#82708,#82709),
 .UNSPECIFIED.,.F.,.F.,(4,2,2,2,2,2,2,2,2,2,2,2,2,2,2,2,2,2,2,2,2,2,2,2,
2,2,2,2,2,2,2,2,2,2,2,2,2,2,2,2,2,2,2,2,2,2,2,2,2,2,2,2,2,2,2,2,2,2,2,2,
2,2,2,2,2,2,2,2,2,2,2,2,2,2,2,2,2,2,2,2,2,2,2,2,2,2,2,2,2,2,2,2,2,2,2,2,
2,2,2,2,2,2,2,2,2,4),(-1.25991862954624,-1.23645521925533,-1.19593125822682,
-1.17294040471037,-1.17008513560625,-1.16870790614013,-1.16763404066988,
-1.16639837265882,-1.16422131132843,-1.15444067563811,-1.10551390453343,
-1.07038842872259,-1.06609282550099,-1.06355136321527,-1.06161049049882,
-1.05953698808853,-1.05628805127453,-1.04597667964511,-1.02941471206419,
-0.996553805928168,-0.982812168797365,-0.975961407222502,-0.975646420836586,
-0.970049533759383,-0.960061038061395,-0.957983607580622,-0.956648423118684,
-0.955577779236245,-0.954311322888828,-0.951992600776219,-0.939846099323988,
-0.88673354569945,-0.858174934537224,-0.854013049428049,-0.85151072086313,
-0.849576244313483,-0.847486387470819,-0.844162406496959,-0.833175585406915,
-0.815089360683986,-0.765144238560623,-0.748663330845422,-0.746024894072714,
-0.744673561711632,-0.743602000668175,-0.742348381533631,-0.740088675562478,
-0.729000855570218,-0.703939740295079,-0.649591388671133,-0.64280991145098,
-0.639962033145629,-0.638172545032308,-0.636208169548954,-0.633484504793157,
-0.626961278490919,-0.597498020898061,-0.552845290504222,-0.536651814362358,
-0.534024869022705,-0.532676044821793,-0.531604703459345,-0.530349293969498,
-0.528081183446334,-0.516848145105593,-0.491226590976862,-0.437702094390137,
-0.43085143562835,-0.427992189719632,-0.426200712641789,-0.424238313712536,
-0.421525052967838,-0.415063422307978,-0.36106306295883,-0.324938440896721,
-0.322081711649332,-0.320704373514572,-0.319630703165592,-0.318395575619336,
-0.316220222184403,-0.306459759801705,-0.257528429502025,-0.222411501761677,
-0.217733600619659,-0.215348296429087,-0.21348532827958,-0.211693434578673,
-0.208570626975831,-0.199301969640913,-0.184975038790322,-0.124596350285011,
-0.112277586646131,-0.110058294587506,-0.108679938431036,-0.107606156828923,
-0.106371671010484,-0.10419928597395,-0.0944824056770145,-0.0455133626512183,
-0.0267278933747515,-0.0187639939523813,-0.00802108700685602,-0.00466632877118399,
-0.00258130087386857,-0.00128118378991342,-0.000628942634120881),
 .UNSPECIFIED.);
#850=B_SPLINE_CURVE_WITH_KNOTS('',3,(#82710,#82711,#82712,#82713,#82714,
#82715,#82716,#82717,#82718,#82719,#82720,#82721,#82722),.UNSPECIFIED.,
 .F.,.F.,(4,3,3,3,4),(-104.372003947921,-104.263735348689,-104.155311094115,
-104.04663122551,-104.0225253952),.UNSPECIFIED.);
#851=B_SPLINE_CURVE_WITH_KNOTS('',3,(#82727,#82728,#82729,#82730,#82731,
#82732,#82733,#82734,#82735,#82736,#82737,#82738,#82739,#82740,#82741,#82742,
#82743,#82744,#82745,#82746,#82747,#82748,#82749,#82750,#82751,#82752,#82753,
#82754,#82755,#82756,#82757,#82758,#82759,#82760,#82761,#82762,#82763,#82764,
#82765,#82766,#82767,#82768,#82769,#82770,#82771,#82772,#82773,#82774,#82775,
#82776,#82777,#82778,#82779,#82780,#82781,#82782,#82783,#82784,#82785,#82786,
#82787,#82788,#82789,#82790,#82791,#82792,#82793,#82794,#82795,#82796,#82797,
#82798,#82799,#82800,#82801,#82802,#82803,#82804,#82805,#82806,#82807,#82808,
#82809,#82810,#82811,#82812,#82813,#82814,#82815,#82816,#82817,#82818,#82819,
#82820,#82821,#82822,#82823,#82824,#82825,#82826,#82827,#82828,#82829,#82830,
#82831,#82832,#82833,#82834,#82835,#82836,#82837,#82838,#82839,#82840,#82841,
#82842,#82843,#82844,#82845,#82846,#82847,#82848,#82849,#82850,#82851,#82852,
#82853,#82854,#82855,#82856,#82857,#82858,#82859,#82860,#82861,#82862,#82863,
#82864,#82865,#82866,#82867,#82868,#82869,#82870,#82871,#82872,#82873,#82874,
#82875,#82876,#82877,#82878,#82879,#82880,#82881,#82882,#82883,#82884,#82885,
#82886,#82887,#82888,#82889,#82890,#82891,#82892,#82893,#82894,#82895,#82896,
#82897,#82898,#82899,#82900,#82901,#82902,#82903,#82904,#82905,#82906,#82907,
#82908,#82909,#82910,#82911,#82912,#82913,#82914,#82915,#82916,#82917,#82918,
#82919,#82920,#82921,#82922,#82923,#82924,#82925,#82926,#82927,#82928,#82929,
#82930,#82931,#82932,#82933,#82934,#82935,#82936,#82937,#82938,#82939,#82940,
#82941,#82942,#82943,#82944,#82945,#82946),.UNSPECIFIED.,.F.,.F.,(4,2,2,
2,2,2,2,2,2,2,2,2,2,2,2,2,2,2,2,2,2,2,2,2,2,2,2,2,2,2,2,2,2,2,2,2,2,2,2,
2,2,2,2,2,2,2,2,2,2,2,2,2,2,2,2,2,2,2,2,2,2,2,2,2,2,2,2,2,2,2,2,2,2,2,2,
2,2,2,2,2,2,2,2,2,2,2,2,2,2,2,2,2,2,2,2,2,2,2,2,2,2,2,2,2,2,2,2,2,2,4),
(-1.40835487586409,-1.37307254728489,-1.33396207527971,-1.33297747199585,
-1.32826978968844,-1.32653031595748,-1.32550498997712,-1.32441215896202,
-1.32290008464717,-1.31930842896567,-1.2801659607581,-1.23134370594005,
-1.22421241397689,-1.22130615321221,-1.21950571385886,-1.21754976278718,
-1.21487490376253,-1.20864154415778,-1.18159616220365,-1.14087028279378,
-1.1182087231562,-1.11535576454838,-1.1139789642684,-1.11290511105388,-1.11166909292598,
-1.10949054261241,-1.09968874450466,-1.05077807375701,-1.01565732978512,
-1.01136167371651,-1.00882015692626,-1.00687922919932,-1.00480565503874,
-1.0015565786924,-0.99124453560085,-0.974681271831154,-0.941818715289484,
-0.928012375820401,-0.921312578881244,-0.905865009656025,-0.903497106721849,
-0.902089528389204,-0.901009372704753,-0.899805921533892,-0.897774110450924,
-0.889883781872256,-0.875166301535708,-0.846103477790437,-0.80369816067887,
-0.799404689283116,-0.796863862784888,-0.794923115277172,-0.792849397165536,
-0.789599392462951,-0.779278473780594,-0.762695310525479,-0.729817092444805,
-0.714521678298897,-0.709793778042114,-0.693941561463135,-0.691328748944117,
-0.689982891872275,-0.688911647877477,-0.687653730721892,-0.685374419074443,
-0.673948878376576,-0.647572475905596,-0.595122290963193,-0.588188791751799,
-0.58531574748797,-0.583521640495918,-0.581561187945153,-0.578859458774007,
-0.572467088305548,-0.526046672481506,-0.484947948273069,-0.480263096992574,
-0.478527315905961,-0.477502865242331,-0.476409860876519,-0.474895739295401,
-0.471290874706858,-0.432949787507504,-0.383317382558082,-0.376221663602101,
-0.373321734996011,-0.371522741093519,-0.369566399214206,-0.366887466226095,
-0.360806593162104,-0.352445785423339,-0.301551359242862,-0.270313240909897,
-0.267401273694885,-0.26601309675877,-0.26493828099778,-0.26371001605091,
-0.261566046985676,-0.252414963091736,-0.20366641682457,-0.167704289702535,
-0.162982355725928,-0.160559557235303,-0.15864067571755,-0.156487801785095,
-0.15425804633715,-0.146612093118065,-0.121083042999811,-0.100337614673059,
-0.0747504805022791),.UNSPECIFIED.);
#852=B_SPLINE_CURVE_WITH_KNOTS('',3,(#82948,#82949,#82950,#82951,#82952,
#82953,#82954,#82955,#82956,#82957,#82958,#82959,#82960,#82961,#82962,#82963,
#82964,#82965,#82966,#82967,#82968,#82969,#82970,#82971,#82972,#82973,#82974,
#82975,#82976,#82977,#82978,#82979,#82980,#82981,#82982,#82983,#82984,#82985,
#82986,#82987,#82988,#82989,#82990,#82991,#82992,#82993,#82994,#82995,#82996,
#82997,#82998,#82999,#83000,#83001,#83002,#83003,#83004,#83005,#83006,#83007,
#83008,#83009,#83010,#83011,#83012,#83013,#83014,#83015,#83016,#83017,#83018,
#83019,#83020,#83021,#83022,#83023,#83024,#83025,#83026,#83027,#83028,#83029,
#83030,#83031,#83032,#83033,#83034,#83035,#83036,#83037,#83038,#83039,#83040,
#83041,#83042,#83043,#83044,#83045,#83046,#83047,#83048,#83049,#83050,#83051,
#83052,#83053,#83054,#83055,#83056,#83057,#83058,#83059,#83060,#83061,#83062,
#83063,#83064,#83065,#83066,#83067,#83068,#83069,#83070,#83071,#83072,#83073,
#83074,#83075,#83076,#83077,#83078,#83079,#83080,#83081,#83082,#83083,#83084,
#83085,#83086,#83087,#83088,#83089,#83090,#83091,#83092,#83093,#83094,#83095,
#83096,#83097,#83098,#83099,#83100,#83101,#83102,#83103,#83104,#83105,#83106,
#83107,#83108,#83109,#83110,#83111,#83112,#83113,#83114,#83115,#83116,#83117,
#83118,#83119,#83120,#83121,#83122,#83123,#83124,#83125,#83126,#83127,#83128),
 .UNSPECIFIED.,.F.,.F.,(4,3,3,3,3,3,3,3,3,3,3,3,3,3,3,3,3,3,3,3,3,3,3,3,
3,3,3,3,3,3,3,3,3,3,3,3,3,3,3,3,3,3,3,3,3,3,3,3,3,3,3,3,3,3,3,3,3,3,3,3,
4),(-104.0225253952,-103.913514251962,-103.878990796035,-103.775596058987,
-103.672354776872,-103.569234811479,-103.46618024327,-103.363157034912,
-103.26013119224,-103.156998425461,-103.053809334052,-102.95043734067,-102.880154346073,
-102.776759609025,-102.67351832691,-102.570398361518,-102.467343793309,
-102.364320584951,-102.261294742279,-102.1581619755,-102.054972884091,-101.951600890709,
-101.881317896111,-101.777923159063,-101.674681876948,-101.571561911556,
-101.468507343347,-101.365484134989,-101.262458292316,-101.159325525538,
-101.056136434129,-100.952764440747,-100.882481446149,-100.779086709101,
-100.675845426986,-100.572725461594,-100.469670893385,-100.366647685027,
-100.263621842355,-100.160489075577,-100.057299984167,-99.9539279907856,
-99.8836449961874,-99.7802502591395,-99.6770089770246,-99.5738890116323,
-99.4708344434235,-99.3678112350658,-99.2647853923932,-99.1616526256151,
-99.0584635342054,-98.9550915408238,-98.8848085462256,-98.7829332776308,
-98.6811932844012,-98.5795525376359,-98.4779751499172,-98.3763829554482,
-98.2747883682234,-98.1730805291731,-98.0888188327624),.UNSPECIFIED.);
#853=B_SPLINE_CURVE_WITH_KNOTS('',3,(#83129,#83130,#83131,#83132,#83133),
 .UNSPECIFIED.,.F.,.F.,(4,1,4),(-98.0888186411165,-97.8859720962637,-97.7379482607811),
 .UNSPECIFIED.);
#854=B_SPLINE_CURVE_WITH_KNOTS('',3,(#83139,#83140,#83141,#83142,#83143,
#83144,#83145,#83146,#83147,#83148,#83149,#83150,#83151,#83152,#83153,#83154,
#83155,#83156,#83157,#83158,#83159,#83160),.UNSPECIFIED.,.F.,.F.,(4,2,2,
2,2,2,2,2,2,2,4),(-0.0750517120858235,-0.0634020277063106,-0.0604359040533312,
-0.0436144771006821,-0.039999553992989,-0.0376361162171469,-0.035722518033051,
-0.0339209987346118,-0.0317709121351228,-0.0286342834260186,-0.000628475014750037),
 .UNSPECIFIED.);
#855=B_SPLINE_CURVE_WITH_KNOTS('',3,(#83161,#83162,#83163,#83164,#83165,
#83166,#83167,#83168,#83169,#83170,#83171,#83172,#83173,#83174,#83175,#83176,
#83177,#83178,#83179,#83180,#83181,#83182,#83183,#83184,#83185,#83186,#83187,
#83188,#83189,#83190,#83191,#83192,#83193,#83194,#83195,#83196,#83197,#83198,
#83199,#83200,#83201,#83202,#83203,#83204,#83205,#83206,#83207,#83208,#83209,
#83210,#83211,#83212,#83213,#83214,#83215,#83216,#83217,#83218,#83219,#83220,
#83221,#83222,#83223,#83224,#83225,#83226,#83227,#83228,#83229,#83230,#83231,
#83232,#83233,#83234,#83235,#83236,#83237,#83238,#83239,#83240,#83241,#83242,
#83243,#83244,#83245,#83246,#83247,#83248,#83249,#83250,#83251,#83252,#83253,
#83254,#83255,#83256,#83257,#83258,#83259,#83260,#83261,#83262,#83263,#83264,
#83265,#83266,#83267,#83268,#83269,#83270,#83271,#83272,#83273,#83274,#83275,
#83276,#83277,#83278,#83279,#83280,#83281,#83282,#83283,#83284,#83285,#83286,
#83287,#83288,#83289,#83290,#83291,#83292,#83293,#83294,#83295,#83296,#83297,
#83298,#83299,#83300,#83301,#83302,#83303,#83304,#83305,#83306,#83307,#83308,
#83309,#83310,#83311,#83312,#83313,#83314,#83315,#83316,#83317,#83318,#83319,
#83320,#83321,#83322,#83323,#83324,#83325,#83326,#83327,#83328,#83329,#83330,
#83331,#83332,#83333,#83334,#83335,#83336,#83337,#83338,#83339,#83340,#83341,
#83342,#83343,#83344,#83345,#83346,#83347,#83348,#83349,#83350,#83351,#83352,
#83353,#83354,#83355,#83356,#83357,#83358,#83359,#83360,#83361,#83362,#83363,
#83364,#83365,#83366,#83367,#83368,#83369,#83370,#83371,#83372,#83373,#83374,
#83375,#83376,#83377,#83378,#83379,#83380,#83381,#83382,#83383,#83384,#83385,
#83386,#83387,#83388),.UNSPECIFIED.,.F.,.F.,(4,2,2,2,2,2,2,2,2,2,2,2,2,
2,2,2,2,2,2,2,2,2,2,2,2,2,2,2,2,2,2,2,2,2,2,2,2,2,2,2,2,2,2,2,2,2,2,2,2,
2,2,2,2,2,2,2,2,2,2,2,2,2,2,2,2,2,2,2,2,2,2,2,2,2,2,2,2,2,2,2,2,2,2,2,2,
2,2,2,2,2,2,2,2,2,2,2,2,2,2,2,2,2,2,2,2,2,2,2,2,2,2,2,2,4),(-2.66755899473746,
-2.62215929206862,-2.60376763862076,-2.5999431884763,-2.59839239054727,
-2.59729261961806,-2.59627719827611,-2.59458840791125,-2.59020935864258,
-2.54255191463499,-2.52187306040523,-2.50663692968774,-2.50017771203682,
-2.49523147431694,-2.49279720522105,-2.49087093917742,-2.48901472241989,
-2.48581672251949,-2.47680447926813,-2.47485034215988,-2.42390161802967,
-2.40007108825067,-2.38930996178348,-2.38706958386249,-2.38582003686064,
-2.38474786226029,-2.38339049507671,-2.38124088461108,-2.37014161526378,
-2.31886838062625,-2.29025511326364,-2.28383242204779,-2.28112537803136,
-2.27916379858666,-2.2773705440319,-2.27450295806638,-2.26760376844898,
-2.21470811541589,-2.18866667499769,-2.17732466173618,-2.17504996632096,
-2.17379296755879,-2.17272152144797,-2.17137415200738,-2.16875471082167,
-2.15275264889233,-2.14725920587629,-2.13282348362516,-2.09992862296215,
-2.08336147074205,-2.07304853117276,-2.06979921902794,-2.06772551199458,
-2.06578447280967,-2.06324282992762,-2.05894703732975,-2.02381486464612,
-1.9748564687468,-1.96513987893544,-1.96296714396137,-1.96173238309113,
-1.96065831835236,-1.95927953159331,-1.95641656331132,-1.93305391234053,
-1.93132070759586,-1.89233867299868,-1.86585625168617,-1.85969299423361,
-1.8570302462541,-1.85507639146389,-1.85327314106256,-1.85035175567705,
-1.8431305892157,-1.7986072322274,-1.78473478757679,-1.7632763083891,-1.75318372698607,
-1.7509856781239,-1.74974535666655,-1.74867205554724,-1.74730153252362,
-1.74510873485366,-1.73333953949705,-1.72962684187481,-1.72236556462697,
-1.67901009008891,-1.66042268288153,-1.64921987459312,-1.64587221244242,
-1.64377679842947,-1.64184352623267,-1.63935164542618,-1.63522643190573,
-1.60809056197531,-1.56616637123774,-1.54954736546721,-1.54098478408796,
-1.53889723340756,-1.53768129444079,-1.53660390223726,-1.53521797734135,
-1.53292427092712,-1.51915032403464,-1.50784479514911,-1.46844818120244,
-1.44187537797694,-1.43570086564228,-1.43303615732892,-1.43108195640327,
-1.42927915351008,-1.42636020670049,-1.41915354266117,-1.40835487586409),
 .UNSPECIFIED.);
#856=B_SPLINE_CURVE_WITH_KNOTS('',3,(#83390,#83391,#83392,#83393,#83394,
#83395,#83396,#83397,#83398,#83399),.UNSPECIFIED.,.F.,.F.,(4,1,1,1,1,1,
1,4),(-97.7379482607811,-96.8871356463018,-95.88829919634,-94.8894627463781,
-93.8906262964162,-92.8917898464543,-91.8929533964925,-91.8056333339369),
 .UNSPECIFIED.);
#857=B_SPLINE_CURVE_WITH_KNOTS('',3,(#83400,#83401,#83402,#83403,#83404,
#83405,#83406,#83407),.UNSPECIFIED.,.F.,.F.,(4,2,2,4),(-2.66776547017807,
-2.61548873906283,-2.59714121576297,-2.59332753526453),.UNSPECIFIED.);
#858=B_SPLINE_CURVE_WITH_KNOTS('',3,(#83412,#83413,#83414,#83415,#83416,
#83417,#83418,#83419,#83420,#83421,#83422,#83423,#83424,#83425,#83426,#83427,
#83428,#83429,#83430,#83431,#83432,#83433,#83434,#83435,#83436,#83437,#83438,
#83439,#83440,#83441,#83442,#83443,#83444,#83445,#83446,#83447,#83448,#83449,
#83450,#83451,#83452,#83453,#83454,#83455,#83456,#83457,#83458,#83459,#83460,
#83461,#83462,#83463,#83464,#83465,#83466,#83467,#83468,#83469,#83470,#83471,
#83472,#83473,#83474,#83475,#83476,#83477,#83478,#83479,#83480,#83481,#83482,
#83483,#83484,#83485,#83486,#83487,#83488,#83489,#83490,#83491,#83492,#83493,
#83494,#83495,#83496,#83497,#83498,#83499,#83500,#83501,#83502,#83503,#83504,
#83505,#83506,#83507,#83508,#83509,#83510,#83511,#83512,#83513,#83514,#83515,
#83516,#83517,#83518,#83519,#83520,#83521,#83522,#83523,#83524,#83525,#83526,
#83527,#83528,#83529,#83530,#83531,#83532,#83533,#83534,#83535,#83536,#83537,
#83538,#83539,#83540,#83541,#83542,#83543,#83544,#83545,#83546,#83547,#83548,
#83549,#83550,#83551,#83552,#83553,#83554,#83555,#83556,#83557,#83558,#83559,
#83560,#83561,#83562,#83563,#83564,#83565,#83566,#83567,#83568,#83569,#83570,
#83571,#83572,#83573,#83574,#83575,#83576,#83577,#83578,#83579,#83580,#83581,
#83582,#83583,#83584,#83585,#83586,#83587,#83588,#83589,#83590,#83591,#83592,
#83593,#83594,#83595,#83596,#83597,#83598,#83599,#83600,#83601,#83602,#83603,
#83604,#83605,#83606,#83607,#83608,#83609,#83610,#83611,#83612,#83613,#83614,
#83615,#83616,#83617,#83618,#83619,#83620,#83621,#83622,#83623,#83624,#83625,
#83626,#83627),.UNSPECIFIED.,.F.,.F.,(4,2,2,2,2,2,2,2,2,2,2,2,2,2,2,2,2,
2,2,2,2,2,2,2,2,2,2,2,2,2,2,2,2,2,2,2,2,2,2,2,2,2,2,2,2,2,2,2,2,2,2,2,2,
2,2,2,2,2,2,2,2,2,2,2,2,2,2,2,2,2,2,2,2,2,2,2,2,2,2,2,2,2,2,2,2,2,2,2,2,
2,2,2,2,2,2,2,2,2,2,2,2,2,2,2,2,2,2,4),(-1.40856932496091,-1.37753543614885,
-1.33437665872906,-1.31573900030673,-1.31200628105946,-1.30960637168692,
-1.30768960262075,-1.30552204984672,-1.30184745235688,-1.28708453682466,
-1.25915948466983,-1.20936256225145,-1.20515960863439,-1.20349963378921,
-1.20248984116764,-1.20138559868045,-1.19981061234075,-1.19583470689363,
-1.17602204218857,-1.14710923645267,-1.10479029204916,-1.10049517751206,
-1.09795393697261,-1.09601319479084,-1.09393979420465,-1.09069093835791,
-1.0803791611172,-1.06381591158189,-1.03095512643785,-1.01703005374874,
-1.01060148456783,-0.995017911007972,-0.992416338826959,-0.991072945979837,
-0.99000190330379,-0.988742175491111,-0.986454345015537,-0.974876083362637,
-0.947885913239259,-0.896303645033721,-0.889312818094277,-0.886430389790255,
-0.884634631904765,-0.882675737586507,-0.87998228355691,-0.873638165877028,
-0.84567906161521,-0.799179368654382,-0.78306850279216,-0.780441838941246,
-0.779093059198093,-0.778021700664243,-0.776766210287376,-0.774497799671683,
-0.763260155420916,-0.737621065911922,-0.684120162797436,-0.677267357996391,
-0.674407723119932,-0.672616149473194,-0.670653763373107,-0.667940738500816,
-0.661480709013897,-0.607538476784662,-0.571348324193975,-0.568493619247127,
-0.567116661797381,-0.566043008375619,-0.564807584295391,-0.562630952565983,
-0.55285224398874,-0.503935138393193,-0.468823866111901,-0.464525059002833,
-0.46198292431333,-0.460042242078175,-0.457969625370875,-0.454723499923555,
-0.44443303529533,-0.42791602817502,-0.371222226226515,-0.35872312561734,
-0.356494177284,-0.355112912291896,-0.354038852235543,-0.35280628338611,
-0.350642590999413,-0.341051024996288,-0.291975395867075,-0.256812360397262,
-0.252513848564328,-0.249971815410669,-0.248031168632203,-0.246240519509763,
-0.243303174701344,-0.235328940876774,-0.223525728322634,-0.190999542299758,
-0.150078407933012,-0.145387637920967,-0.143651113228751,-0.142626620497403,
-0.141533908642349,-0.140020743409252,-0.136420703033798,-0.0985274293922583,
-0.075735778076427,-0.0750517120858235),.UNSPECIFIED.);
#859=B_SPLINE_CURVE_WITH_KNOTS('',3,(#83628,#83629,#83630,#83631,#83632,
#83633,#83634,#83635,#83636,#83637,#83638,#83639,#83640,#83641,#83642,#83643,
#83644,#83645,#83646,#83647,#83648,#83649,#83650,#83651,#83652,#83653,#83654,
#83655,#83656,#83657,#83658,#83659,#83660,#83661,#83662,#83663,#83664,#83665,
#83666,#83667,#83668,#83669,#83670,#83671,#83672,#83673,#83674,#83675,#83676,
#83677,#83678,#83679,#83680,#83681,#83682,#83683,#83684,#83685,#83686,#83687,
#83688,#83689,#83690,#83691,#83692,#83693,#83694,#83695,#83696,#83697,#83698,
#83699,#83700,#83701,#83702,#83703,#83704,#83705,#83706,#83707,#83708,#83709,
#83710,#83711,#83712,#83713,#83714,#83715,#83716,#83717,#83718,#83719,#83720,
#83721,#83722,#83723,#83724,#83725,#83726,#83727,#83728,#83729,#83730,#83731,
#83732,#83733,#83734,#83735,#83736,#83737,#83738,#83739,#83740,#83741,#83742,
#83743,#83744,#83745,#83746,#83747,#83748,#83749,#83750,#83751,#83752,#83753,
#83754,#83755,#83756,#83757,#83758,#83759,#83760,#83761,#83762,#83763,#83764,
#83765,#83766,#83767,#83768,#83769,#83770,#83771,#83772,#83773,#83774,#83775,
#83776,#83777,#83778,#83779,#83780,#83781,#83782,#83783,#83784,#83785,#83786,
#83787,#83788,#83789,#83790,#83791,#83792,#83793,#83794,#83795,#83796,#83797,
#83798,#83799,#83800,#83801,#83802,#83803,#83804,#83805,#83806,#83807,#83808,
#83809,#83810,#83811,#83812,#83813,#83814,#83815,#83816,#83817,#83818,#83819,
#83820,#83821,#83822,#83823,#83824,#83825,#83826,#83827,#83828,#83829,#83830,
#83831,#83832,#83833,#83834,#83835,#83836,#83837,#83838,#83839,#83840,#83841,
#83842,#83843,#83844,#83845,#83846,#83847,#83848,#83849,#83850,#83851,#83852,
#83853,#83854,#83855,#83856,#83857,#83858,#83859,#83860,#83861,#83862,#83863,
#83864,#83865,#83866,#83867,#83868,#83869,#83870,#83871,#83872,#83873,#83874,
#83875,#83876,#83877,#83878,#83879,#83880,#83881,#83882,#83883,#83884,#83885,
#83886,#83887,#83888,#83889,#83890,#83891,#83892,#83893,#83894,#83895,#83896,
#83897,#83898,#83899),.UNSPECIFIED.,.F.,.F.,(4,2,2,2,2,2,2,2,2,2,2,2,2,
2,2,2,2,2,2,2,2,2,2,2,2,2,2,2,2,2,2,2,2,2,2,2,2,2,2,2,2,2,2,2,2,2,2,2,2,
2,2,2,2,2,2,2,2,2,2,2,2,2,2,2,2,2,2,2,2,2,2,2,2,2,2,2,2,2,2,2,2,2,2,2,2,
2,2,2,2,2,2,2,2,2,2,2,2,2,2,2,2,2,2,2,2,2,2,2,2,2,2,2,2,2,2,2,2,2,2,2,2,
2,2,2,2,2,2,2,2,2,2,2,2,2,2,4),(-2.59332753526453,-2.58604272140604,-2.58270693816439,
-2.5806146222872,-2.57868125454311,-2.57618511262564,-2.57204387356041,
-2.54424358251689,-2.5020144615368,-2.48613393383352,-2.48061668953957,
-2.47798287951046,-2.47587129426084,-2.4746488810723,-2.47464532648293,
-2.47464175810497,-2.47463817596284,-2.47463457982111,-2.47463071128106,
-2.47462677538248,-2.47462277065502,-2.47461869567567,-2.47461454885354,
-2.47461032863313,-2.47460603362575,-2.47460166216701,-2.47459721247322,
-2.47459268293298,-2.47458807165657,-2.4745833768235,-2.47457859663824,
-2.47457372915854,-2.47354854823527,-2.47217419824068,-2.46933247020453,
-2.4324211405773,-2.4008118662466,-2.3842491625337,-2.37393905210402,-2.37069066332947,
-2.36861755328192,-2.36667707829501,-2.36413618198753,-2.35984166871282,
-2.32472230221683,-2.27578630969899,-2.26606285126058,-2.26389008000958,
-2.26265553054566,-2.26158179848073,-2.26020363344686,-2.25734262753862,
-2.23404573343154,-2.22174771777207,-2.18886060901367,-2.17229758466922,
-2.16198714947012,-2.15873859178091,-2.15666535793356,-2.15472475582895,
-2.15218367685695,-2.14788881851329,-2.11276178546471,-2.06380576078331,
-2.05410161024298,-2.05193007164809,-2.05069574502374,-2.04962190040874,
-2.04824318995788,-2.04537966827013,-2.00941117954529,-1.95514326922882,
-1.94873698692295,-1.94603301867958,-1.94407227005156,-1.94227881183604,
-1.93940880109859,-1.93249290780156,-1.87984542234686,-1.85364247756406,
-1.84226041877107,-1.83998373772502,-1.83872645003023,-1.83765524751299,
-1.8363088075184,-1.83369300264878,-1.81775261430373,-1.81207173027847,
-1.76791434511493,-1.74936380567546,-1.73817766206365,-1.73483233658984,
-1.73273779450941,-1.7308049254761,-1.7283130033667,-1.7241865081184,-1.69696510608635,
-1.65487193717336,-1.63845567834265,-1.62996335994081,-1.62788176391822,
-1.62666734280498,-1.62558997700872,-1.62420238242251,-1.62190237600633,
-1.60798933621419,-1.60636834810441,-1.60500975276388,-1.59754427077589,
-1.58574630989523,-1.55288290017062,-1.53634916157398,-1.52605188088118,
-1.52280476471924,-1.52073180074514,-1.5187909944066,-1.51624898862964,
-1.51195108538526,-1.47659208651493,-1.42743051949544,-1.4181151048594,
-1.4159709222603,-1.41474259569936,-1.41366777097751,-1.41227963111758,
-1.40936793066897,-1.37753518108014,-1.33437642004894,-1.31573877104263,
-1.31200605425729,-1.30960614657258,-1.30768937892502,-1.30552182783276,
-1.30184723338871,-1.28708433298769,-1.25997080151201),.UNSPECIFIED.);
#860=B_SPLINE_CURVE_WITH_KNOTS('',3,(#83905,#83906,#83907,#83908,#83909),
 .UNSPECIFIED.,.F.,.F.,(4,1,4),(82.6397394574315,82.9034253468356,82.9907454093913),
 .UNSPECIFIED.);
#861=B_SPLINE_CURVE_WITH_KNOTS('',3,(#83910,#83911,#83912,#83913,#83914,
#83915,#83916,#83917,#83918,#83919,#83920,#83921,#83922,#83923,#83924,#83925,
#83926,#83927,#83928,#83929,#83930,#83931,#83932,#83933,#83934,#83935,#83936,
#83937,#83938,#83939,#83940,#83941,#83942,#83943,#83944,#83945,#83946,#83947,
#83948,#83949,#83950,#83951,#83952,#83953,#83954,#83955,#83956,#83957,#83958,
#83959,#83960,#83961,#83962,#83963,#83964,#83965,#83966,#83967,#83968,#83969,
#83970,#83971,#83972,#83973,#83974,#83975,#83976,#83977,#83978,#83979,#83980,
#83981,#83982,#83983,#83984,#83985,#83986,#83987,#83988,#83989,#83990,#83991,
#83992,#83993,#83994,#83995,#83996,#83997,#83998,#83999,#84000,#84001,#84002,
#84003,#84004,#84005,#84006,#84007,#84008,#84009,#84010,#84011,#84012,#84013,
#84014,#84015,#84016,#84017,#84018,#84019,#84020,#84021,#84022,#84023,#84024,
#84025,#84026,#84027,#84028,#84029,#84030,#84031,#84032,#84033,#84034,#84035,
#84036,#84037,#84038,#84039,#84040,#84041,#84042,#84043,#84044,#84045,#84046,
#84047,#84048,#84049,#84050,#84051,#84052,#84053,#84054,#84055,#84056,#84057,
#84058,#84059,#84060,#84061,#84062,#84063,#84064,#84065,#84066,#84067,#84068,
#84069,#84070,#84071,#84072,#84073,#84074,#84075,#84076,#84077,#84078,#84079,
#84080,#84081,#84082,#84083,#84084,#84085,#84086,#84087,#84088,#84089,#84090,
#84091,#84092,#84093,#84094,#84095,#84096,#84097,#84098,#84099,#84100,#84101,
#84102,#84103,#84104,#84105,#84106,#84107,#84108,#84109,#84110,#84111,#84112,
#84113,#84114,#84115,#84116,#84117,#84118,#84119,#84120,#84121,#84122,#84123,
#84124,#84125,#84126,#84127,#84128,#84129,#84130,#84131,#84132,#84133,#84134,
#84135,#84136,#84137,#84138,#84139,#84140,#84141,#84142,#84143,#84144,#84145,
#84146,#84147,#84148,#84149,#84150,#84151,#84152,#84153,#84154,#84155,#84156,
#84157,#84158,#84159,#84160,#84161,#84162,#84163,#84164,#84165),
 .UNSPECIFIED.,.F.,.F.,(4,2,2,2,2,2,2,2,2,2,2,2,2,2,2,2,2,2,2,2,2,2,2,2,
2,2,2,2,2,2,2,2,2,2,2,2,2,2,2,2,2,2,2,2,2,2,2,2,2,2,2,2,2,2,2,2,2,2,2,2,
2,2,2,2,2,2,2,2,2,2,2,2,2,2,2,2,2,2,2,2,2,2,2,2,2,2,2,2,2,2,2,2,2,2,2,2,
2,2,2,2,2,2,2,2,2,2,2,2,2,2,2,2,2,2,2,2,2,2,2,2,2,2,2,2,2,2,2,4),(-2.66783332377647,
-2.61564214598672,-2.59723508098817,-2.58611069517746,-2.58277199335766,
-2.58067893953301,-2.57874563411728,-2.57625061549819,-2.57211350181238,
-2.54447923335572,-2.50218480438026,-2.48622223875291,-2.48068593668643,
-2.47804556179293,-2.47592965463349,-2.47470621549526,-2.47470267000306,
-2.47469911096232,-2.47469553816781,-2.47469195165705,-2.47468835133991,
-2.47468446315151,-2.47468050715029,-2.47467648191082,-2.47467238588093,
-2.47466821771319,-2.47466397579209,-2.47465965849242,-2.47465526417203,
-2.47465079116621,-2.47464623767288,-2.47464160202744,-2.47463688241049,
-2.47463207674742,-2.47360824688145,-2.47223647282876,-2.46940783145152,
-2.43186080881884,-2.40255942178994,-2.37839554315062,-2.37252897073714,
-2.36991916296777,-2.36797474773041,-2.36615912463568,-2.36365902174291,
-2.35727484377884,-2.29920250318749,-2.27659273967936,-2.26617046426924,
-2.2639514909605,-2.26270677441483,-2.26163431559197,-2.26027087279878,
-2.25748458055384,-2.23740819260861,-2.19455466466653,-2.16700963873722,
-2.16071622685985,-2.15803143271454,-2.1560740845448,-2.15427644663709,
-2.15138372890445,-2.14433095227195,-2.09387723167345,-2.05630415343087,
-2.05272440615339,-2.05121460198596,-2.05012238409171,-2.04909681596941,
-2.04735518562612,-2.04263149798945,-2.00238929811358,-1.95513209844072,
-1.94873720900797,-1.94603516014328,-1.94407474979468,-1.94228087443214,
-1.93940861073604,-1.93247909119843,-1.88001945152264,-1.85368423493556,
-1.84226877993537,-1.83999018882601,-1.83873248222893,-1.83766130778611,
-1.83631539250319,-1.83370204194143,-1.81782624216145,-1.81303239894487,
-1.76784553711486,-1.74934089879086,-1.73817446959149,-1.7348312422891,
-1.73273716392597,-1.73080414496727,-1.72831122132682,-1.72418131817348,
-1.69682711648576,-1.65453192776829,-1.63835940965027,-1.62995128134607,
-1.62787644307332,-1.62666352117122,-1.62558582731251,-1.62419566345088,
-1.6218869252826,-1.60779514032835,-1.60650289106458,-1.60500052111857,
-1.59754568222509,-1.58574671518815,-1.55288327876266,-1.53634952170758,
-1.52605223069659,-1.52280511182253,-1.52073214624075,-1.51879133848219,
-1.51624933096568,-1.5119514250411,-1.47659242780067,-1.42743081628971,
-1.41811539257215,-1.41597120822893,-1.41474288072132,-1.41366805520194,
-1.41227991434118,-1.40936821188941,-1.40856932496091),.UNSPECIFIED.);
#862=B_SPLINE_CURVE_WITH_KNOTS('',3,(#84167,#84168,#84169,#84170,#84171,
#84172,#84173,#84174,#84175,#84176,#84177,#84178,#84179,#84180,#84181,#84182,
#84183,#84184,#84185,#84186,#84187,#84188,#84189,#84190,#84191,#84192,#84193,
#84194,#84195,#84196,#84197,#84198,#84199,#84200,#84201,#84202,#84203,#84204,
#84205,#84206,#84207,#84208,#84209,#84210,#84211,#84212,#84213,#84214,#84215,
#84216,#84217,#84218,#84219,#84220,#84221,#84222,#84223,#84224,#84225,#84226,
#84227,#84228,#84229,#84230,#84231,#84232,#84233,#84234,#84235,#84236,#84237,
#84238,#84239,#84240,#84241,#84242,#84243,#84244,#84245,#84246,#84247,#84248,
#84249,#84250,#84251,#84252,#84253,#84254,#84255,#84256,#84257,#84258,#84259,
#84260,#84261,#84262,#84263,#84264,#84265,#84266,#84267,#84268,#84269,#84270,
#84271,#84272,#84273,#84274,#84275,#84276,#84277,#84278,#84279,#84280,#84281,
#84282,#84283,#84284,#84285,#84286,#84287,#84288,#84289,#84290,#84291,#84292,
#84293,#84294,#84295,#84296,#84297,#84298,#84299,#84300,#84301,#84302,#84303,
#84304,#84305,#84306,#84307,#84308,#84309,#84310,#84311,#84312,#84313,#84314,
#84315,#84316,#84317,#84318,#84319,#84320,#84321,#84322,#84323,#84324,#84325,
#84326,#84327,#84328,#84329,#84330,#84331,#84332,#84333,#84334,#84335,#84336,
#84337,#84338,#84339,#84340,#84341,#84342,#84343,#84344,#84345,#84346,#84347,
#84348,#84349,#84350,#84351,#84352,#84353,#84354,#84355,#84356,#84357,#84358,
#84359,#84360,#84361,#84362,#84363,#84364,#84365,#84366,#84367,#84368,#84369,
#84370,#84371,#84372,#84373,#84374,#84375,#84376,#84377,#84378,#84379,#84380,
#84381,#84382),.UNSPECIFIED.,.F.,.F.,(4,2,2,2,2,2,2,2,2,2,2,2,2,2,2,2,2,
2,2,2,2,2,2,2,2,2,2,2,2,2,2,2,2,2,2,2,2,2,2,2,2,2,2,2,2,2,2,2,2,2,2,2,2,
2,2,2,2,2,2,2,2,2,2,2,2,2,2,2,2,2,2,2,2,2,2,2,2,2,2,2,2,2,2,2,2,2,2,2,2,
2,2,2,2,2,2,2,2,2,2,2,2,2,2,2,2,2,2,4),(-1.25997080151201,-1.25915931516951,
-1.20936239081794,-1.20515944182619,-1.20349946847035,-1.20248967664927,
-1.20138543494635,-1.19981044958039,-1.19583454584559,-1.17602188455216,
-1.14710910079787,-1.10479018260538,-1.10049507090556,-1.09795383215206,
-1.09601309139939,-1.09393969240468,-1.09069083919058,-1.08037907156495,
-1.06381583893288,-1.03095507917741,-1.01703065887685,-1.01060068296542,
-0.995017815824003,-0.992416275187708,-0.991072889737169,-0.990001848249544,
-0.988742116367917,-0.986454264495089,-0.974875597907575,-0.947883774590537,
-0.896303860887372,-0.8893128934105,-0.886430443104705,-0.884634682141149,
-0.882675792949477,-0.879982361414452,-0.873638368776958,-0.845680281583233,
-0.799190527300124,-0.783069970251435,-0.78044247775776,-0.779093520367573,
-0.778022150678918,-0.776766797655267,-0.774499016245602,-0.76327220566548,
-0.737675201382725,-0.684113304354058,-0.677265455766238,-0.674406638539597,
-0.672615213852687,-0.670652697978992,-0.667938954844861,-0.661474646410106,
-0.607384724107681,-0.571356490359434,-0.568496370848481,-0.567118351271025,
-0.566044597040419,-0.564809877739583,-0.562636449235622,-0.552904502334806,
-0.503947924152347,-0.468806688720381,-0.464517287132083,-0.461977879737483,
-0.460037645928899,-0.457963923376715,-0.454712755279172,-0.444378370302155,
-0.427764255914947,-0.371064364763453,-0.358708582439002,-0.356487302632965,
-0.355108350939898,-0.354034517687593,-0.352800437326769,-0.350629874308427,
-0.34093930465962,-0.29194827702703,-0.256811872620156,-0.25251362990003,
-0.249971674950569,-0.248031041291889,-0.246240392883459,-0.243302951930731,
-0.235328044223839,-0.223523527455889,-0.190998694030786,-0.150078466355593,
-0.145387650131162,-0.143651118608479,-0.142626624664606,-0.141533913915671,
-0.14002075414421,-0.136420744922919,-0.0985306498520224,-0.0757357801641774,
-0.0634020321937908,-0.0604357376939238,-0.0436144584964585,-0.0399995456229471,
-0.0376361112330499,-0.0357225135970766,-0.0339209942593315,-0.0317709059834869,
-0.0286342728390913,-0.000628476974914811),.UNSPECIFIED.);
#863=B_SPLINE_CURVE_WITH_KNOTS('',3,(#84383,#84384,#84385,#84386,#84387,
#84388,#84389,#84390,#84391,#84392,#84393,#84394,#84395,#84396,#84397,#84398,
#84399,#84400),.UNSPECIFIED.,.F.,.F.,(4,2,2,2,2,2,2,2,4),(-2.6675682063545,
-2.62399424995869,-2.60401305473231,-2.60001889487262,-2.59844083514121,
-2.59733583662049,-2.59632642690663,-2.59466920107051,-2.59342127676457),
 .UNSPECIFIED.);
#864=B_SPLINE_CURVE_WITH_KNOTS('',3,(#84406,#84407,#84408,#84409,#84410,
#84411,#84412,#84413,#84414,#84415,#84416,#84417,#84418),.UNSPECIFIED.,
 .F.,.F.,(4,3,3,3,4),(76.3573194355999,76.4589087585747,76.5605127542266,
76.6622237698669,76.7075599105224),.UNSPECIFIED.);
#865=B_SPLINE_CURVE_WITH_KNOTS('',3,(#84419,#84420,#84421,#84422,#84423,
#84424,#84425,#84426,#84427,#84428),.UNSPECIFIED.,.F.,.F.,(4,1,1,1,1,1,
1,4),(76.7075601022117,76.9104066470643,77.9092430970262,78.9080795469881,
79.90691599695,80.9057524469119,81.9045888968737,82.6397394574315),
 .UNSPECIFIED.);
#866=B_SPLINE_CURVE_WITH_KNOTS('',3,(#84429,#84430,#84431,#84432,#84433,
#84434,#84435,#84436,#84437,#84438,#84439,#84440,#84441,#84442,#84443,#84444,
#84445,#84446,#84447,#84448,#84449,#84450,#84451,#84452,#84453,#84454,#84455,
#84456,#84457,#84458,#84459,#84460,#84461,#84462,#84463,#84464,#84465,#84466,
#84467,#84468,#84469,#84470,#84471,#84472,#84473,#84474,#84475,#84476,#84477,
#84478,#84479,#84480,#84481,#84482,#84483,#84484,#84485,#84486,#84487,#84488,
#84489,#84490,#84491,#84492,#84493,#84494,#84495,#84496,#84497,#84498,#84499,
#84500,#84501,#84502,#84503,#84504,#84505,#84506,#84507,#84508,#84509,#84510,
#84511,#84512,#84513,#84514,#84515,#84516,#84517,#84518,#84519,#84520,#84521,
#84522,#84523,#84524,#84525,#84526,#84527,#84528,#84529,#84530,#84531,#84532,
#84533,#84534,#84535,#84536,#84537,#84538,#84539,#84540,#84541,#84542,#84543,
#84544,#84545,#84546,#84547,#84548,#84549,#84550,#84551,#84552,#84553,#84554,
#84555,#84556,#84557,#84558,#84559,#84560,#84561,#84562,#84563,#84564,#84565,
#84566,#84567,#84568,#84569,#84570,#84571,#84572,#84573,#84574,#84575,#84576,
#84577,#84578,#84579,#84580,#84581,#84582,#84583,#84584,#84585,#84586,#84587,
#84588,#84589,#84590,#84591,#84592,#84593,#84594,#84595,#84596,#84597,#84598,
#84599,#84600,#84601,#84602,#84603,#84604,#84605,#84606,#84607,#84608,#84609,
#84610,#84611,#84612,#84613,#84614,#84615,#84616,#84617,#84618,#84619,#84620,
#84621,#84622,#84623,#84624,#84625,#84626,#84627,#84628,#84629,#84630,#84631,
#84632,#84633,#84634,#84635,#84636,#84637,#84638,#84639,#84640,#84641,#84642,
#84643,#84644,#84645,#84646,#84647,#84648,#84649,#84650,#84651,#84652,#84653,
#84654,#84655,#84656),.UNSPECIFIED.,.F.,.F.,(4,2,2,2,2,2,2,2,2,2,2,2,2,
2,2,2,2,2,2,2,2,2,2,2,2,2,2,2,2,2,2,2,2,2,2,2,2,2,2,2,2,2,2,2,2,2,2,2,2,
2,2,2,2,2,2,2,2,2,2,2,2,2,2,2,2,2,2,2,2,2,2,2,2,2,2,2,2,2,2,2,2,2,2,2,2,
2,2,2,2,2,2,2,2,2,2,2,2,2,2,2,2,2,2,2,2,2,2,2,2,2,2,2,2,4),(-2.59342127676457,
-2.59048347284373,-2.54045199528121,-2.51630178484054,-2.50447831747976,
-2.49650002328404,-2.49355707467113,-2.49176590198081,-2.48982514440233,
-2.48728500586137,-2.48299429910268,-2.44777540686383,-2.39856697908379,
-2.3891424325095,-2.38699017674455,-2.38575994222461,-2.38468521307211,
-2.38329952089089,-2.38040111992613,-2.35385739992858,-2.31526623638961,
-2.29654057056957,-2.28527861604887,-2.28192471693209,-2.27982794224699,
-2.27789513903704,-2.27540626891932,-2.27129123399137,-2.24455521972296,
-2.20210370055799,-2.18556312888556,-2.17702741818053,-2.17494201465344,
-2.17372656058519,-2.172649081184,-2.1712623768787,-2.16896599724637,-2.15513638327683,
-2.10779708797665,-2.07839186059568,-2.07187523012424,-2.06915229639498,
-2.06718772501885,-2.06539756810838,-2.06254755632007,-2.05575554413522,
-2.0015313401453,-1.97640103482375,-1.96529343999646,-1.96303224305336,
-1.96177812980237,-1.96070635366049,-1.95935500803608,-1.95671731284662,
-1.94026815262134,-1.93129592700923,-1.892333429793,-1.86585500528528,-1.85969224367934,
-1.85702958086473,-1.85507573992727,-1.85327246813406,-1.85035097167035,
-1.84312915331335,-1.79883075419771,-1.78472735817278,-1.76327449280604,
-1.75318355352458,-1.75098561310118,-1.74974531556408,-1.74867201157841,
-1.7473014542876,-1.74510854310032,-1.73333758204521,-1.72962677565314,
-1.72236564461493,-1.67901010743369,-1.6604227014912,-1.64921989415206,
-1.64587223247618,-1.64377681881014,-1.64184354696978,-1.63935166667531,
-1.63522645412308,-1.60809060366594,-1.56616641310786,-1.54954739157589,
-1.54098480514965,-1.53889725431586,-1.53768131544922,-1.53660392346626,
-1.53521799903576,-1.53292429377116,-1.51915036506596,-1.50784474710706,
-1.46844818572822,-1.44187539589865,-1.43570088566117,-1.43303617799437,
-1.4310819774494,-1.42927917484296,-1.42636022835657,-1.41915356445291,
-1.37307258371222,-1.33396209739049,-1.33297755094329,-1.32826982515185,
-1.32653034500397,-1.32550501788735,-1.32441218791099,-1.32290011871591,
-1.31930849215528,-1.28017021908768,-1.25968440107285),.UNSPECIFIED.);
#867=B_SPLINE_CURVE_WITH_KNOTS('',3,(#84662,#84663,#84664,#84665,#84666,
#84667,#84668,#84669,#84670,#84671,#84672,#84673,#84674,#84675,#84676,#84677),
 .UNSPECIFIED.,.F.,.F.,(4,2,2,2,2,2,2,4),(-0.0749587606043023,-0.0267279161832551,
-0.0187640096720314,-0.00802108930702553,-0.00466632912088836,-0.00258130053910898,
-0.00128118358441392,-0.000628940636314346),.UNSPECIFIED.);
#868=B_SPLINE_CURVE_WITH_KNOTS('',3,(#84678,#84679,#84680,#84681,#84682,
#84683,#84684,#84685,#84686,#84687,#84688,#84689,#84690,#84691,#84692,#84693,
#84694,#84695,#84696,#84697,#84698,#84699,#84700,#84701,#84702,#84703,#84704,
#84705,#84706,#84707,#84708,#84709,#84710,#84711,#84712,#84713,#84714,#84715,
#84716,#84717,#84718,#84719,#84720,#84721,#84722,#84723,#84724,#84725,#84726,
#84727,#84728,#84729,#84730,#84731,#84732,#84733,#84734,#84735,#84736,#84737,
#84738,#84739,#84740,#84741,#84742,#84743,#84744,#84745,#84746,#84747,#84748,
#84749,#84750,#84751,#84752,#84753,#84754,#84755,#84756,#84757,#84758,#84759,
#84760,#84761,#84762,#84763,#84764,#84765,#84766,#84767,#84768,#84769,#84770,
#84771,#84772,#84773,#84774,#84775,#84776,#84777,#84778,#84779,#84780,#84781,
#84782,#84783,#84784,#84785,#84786,#84787,#84788,#84789,#84790,#84791,#84792,
#84793,#84794,#84795,#84796,#84797,#84798,#84799,#84800,#84801,#84802,#84803,
#84804,#84805,#84806,#84807,#84808,#84809,#84810,#84811,#84812,#84813,#84814,
#84815,#84816,#84817,#84818,#84819,#84820,#84821,#84822,#84823,#84824,#84825,
#84826,#84827,#84828,#84829,#84830,#84831,#84832,#84833,#84834,#84835,#84836,
#84837,#84838,#84839,#84840,#84841,#84842,#84843,#84844,#84845,#84846,#84847,
#84848,#84849,#84850,#84851,#84852,#84853,#84854,#84855,#84856,#84857,#84858),
 .UNSPECIFIED.,.F.,.F.,(4,3,3,3,3,3,3,3,3,3,3,3,3,3,3,3,3,3,3,3,3,3,3,3,
3,3,3,3,3,3,3,3,3,3,3,3,3,3,3,3,3,3,3,3,3,3,3,3,3,3,3,3,3,3,3,3,3,3,3,3,
4),(70.4243747954073,70.5325790413761,70.6410991164245,70.7497863837826,
70.8587740112805,70.9173879472931,71.020782684341,71.124023966456,71.2271439318483,
71.3301985000572,71.433221708415,71.5362475510875,71.6393803178656,71.7425694092754,
71.8459414026571,71.916224397255,72.0196191343029,72.1228604164179,72.2259803818102,
72.3290349500191,72.4320581583768,72.5350840010493,72.6382167678273,72.7414058592371,
72.8447778526187,72.9150608472168,73.0184555842647,73.1216968663798,73.2248168317721,
73.327871399981,73.4308946083388,73.5339204510113,73.6370532177894,73.7402423091992,
73.8436143025809,73.9138972971787,74.0172920342266,74.1205333163417,74.2236532817339,
74.3267078499429,74.4297310583006,74.5327569009731,74.6358896677512,74.739078759161,
74.8424507525426,74.9127337471406,75.0161284841885,75.1193697663036,75.2224897316958,
75.3255442999048,75.4285675082625,75.531593350935,75.6347261177131,75.7379152091229,
75.8412872025045,75.9115701971025,76.0134810050448,76.1152211478867,76.2168630906399,
76.3184433457415,76.3573194355999),.UNSPECIFIED.);
#869=B_SPLINE_CURVE_WITH_KNOTS('',3,(#84860,#84861,#84862,#84863,#84864,
#84865,#84866,#84867,#84868,#84869,#84870,#84871,#84872,#84873,#84874,#84875,
#84876,#84877,#84878,#84879,#84880,#84881,#84882,#84883,#84884,#84885,#84886,
#84887,#84888,#84889,#84890,#84891,#84892,#84893,#84894,#84895,#84896,#84897,
#84898,#84899,#84900,#84901,#84902,#84903,#84904,#84905,#84906,#84907,#84908,
#84909,#84910,#84911,#84912,#84913,#84914,#84915,#84916,#84917,#84918,#84919,
#84920,#84921,#84922,#84923,#84924,#84925,#84926,#84927,#84928,#84929,#84930,
#84931,#84932,#84933,#84934,#84935,#84936,#84937,#84938,#84939,#84940,#84941,
#84942,#84943,#84944,#84945,#84946,#84947,#84948,#84949,#84950,#84951,#84952,
#84953,#84954,#84955,#84956,#84957,#84958,#84959,#84960,#84961,#84962,#84963,
#84964,#84965,#84966,#84967,#84968,#84969,#84970,#84971,#84972,#84973,#84974,
#84975,#84976,#84977,#84978,#84979,#84980,#84981,#84982,#84983,#84984,#84985,
#84986,#84987,#84988,#84989,#84990,#84991,#84992,#84993,#84994,#84995,#84996,
#84997,#84998,#84999,#85000,#85001,#85002,#85003,#85004,#85005,#85006,#85007,
#85008,#85009,#85010,#85011,#85012,#85013,#85014,#85015,#85016,#85017,#85018,
#85019,#85020,#85021,#85022,#85023,#85024,#85025,#85026,#85027,#85028,#85029,
#85030,#85031,#85032,#85033,#85034,#85035,#85036,#85037,#85038,#85039,#85040,
#85041,#85042,#85043,#85044,#85045,#85046,#85047,#85048,#85049,#85050,#85051,
#85052,#85053,#85054,#85055,#85056,#85057,#85058,#85059,#85060,#85061,#85062,
#85063,#85064,#85065,#85066,#85067,#85068,#85069,#85070,#85071,#85072,#85073,
#85074,#85075),.UNSPECIFIED.,.F.,.F.,(4,2,2,2,2,2,2,2,2,2,2,2,2,2,2,2,2,
2,2,2,2,2,2,2,2,2,2,2,2,2,2,2,2,2,2,2,2,2,2,2,2,2,2,2,2,2,2,2,2,2,2,2,2,
2,2,2,2,2,2,2,2,2,2,2,2,2,2,2,2,2,2,2,2,2,2,2,2,2,2,2,2,2,2,2,2,2,2,2,2,
2,2,2,2,2,2,2,2,2,2,2,2,2,2,2,2,2,2,4),(-1.25968440107285,-1.23134347578101,
-1.22421236147874,-1.22130613077246,-1.21950569718235,-1.21754974221429,
-1.214874859563,-1.20864136135389,-1.18159485028042,-1.14086664256386,-1.11820860043456,
-1.11535572835216,-1.11397894521092,-1.11290509378181,-1.11166906463371,
-1.10949046358634,-1.09968791701672,-1.05077788475576,-1.0156573381461,
-1.01136168517331,-1.00882016949855,-1.00687924221377,-1.00480566813094,
-1.00155659108614,-0.991244538944737,-0.97468125440176,-0.941818681000237,
-0.92801074099284,-0.921314654636271,-0.905865157336135,-0.903497179120168,
-0.902089578970233,-0.901009420370377,-0.899805981254557,-0.89777422375533,
-0.889884513358211,-0.875168727792606,-0.846104339448585,-0.803698147926956,
-0.799404688600541,-0.796863865827195,-0.794923119199462,-0.792849400123064,
-0.789599389932939,-0.77927842035718,-0.76269514373061,-0.729816832146161,
-0.714514095931957,-0.709793811429688,-0.693941568281681,-0.691328755516341,
-0.68998289852579,-0.68891165470866,-0.687653737904237,-0.685374427258513,
-0.673948899363318,-0.647572546076294,-0.595122289395258,-0.588188795527061,
-0.58531575244097,-0.583521645885682,-0.581561193574165,-0.578859464301349,
-0.572467091586332,-0.52604566064621,-0.484947992336852,-0.480263111631424,
-0.478527326250482,-0.477502874864194,-0.476409871273696,-0.474895753303722,
-0.471290909056834,-0.432951879871835,-0.383317243140413,-0.376221625973913,
-0.373321714677207,-0.371522724177452,-0.369566380190154,-0.366887433827155,
-0.360806482143914,-0.352445538208922,-0.301550797636007,-0.270313243057044,
-0.267401275346587,-0.266013098458514,-0.264938282866957,-0.26371001827139,
-0.261566050199208,-0.252414976638071,-0.203666464120236,-0.167704290948247,
-0.162982357055917,-0.160559558829926,-0.15864067763351,-0.156487804181213,
-0.154258049270772,-0.146612099116105,-0.121083046665255,-0.100337619252734,
-0.0610229402433785,-0.0562870055113607,-0.0545435823234888,-0.0535177065565094,
-0.0524257940207308,-0.0509174412395485,-0.0492296228409805,-0.0462824128736715,
-0.000629120905446686),.UNSPECIFIED.);
#870=B_SPLINE_CURVE_WITH_KNOTS('',3,(#85076,#85077,#85078,#85079,#85080,
#85081,#85082,#85083,#85084,#85085,#85086,#85087,#85088),.UNSPECIFIED.,
 .F.,.F.,(4,3,3,3,4),(-66.6728921052185,-66.5709585796818,-66.4690950147619,
-66.3672509448715,-66.322858757962),.UNSPECIFIED.);
#871=B_SPLINE_CURVE_WITH_KNOTS('',3,(#85093,#85094,#85095,#85096,#85097,
#85098,#85099,#85100,#85101,#85102,#85103,#85104,#85105,#85106,#85107,#85108,
#85109,#85110,#85111,#85112,#85113,#85114,#85115,#85116,#85117,#85118,#85119,
#85120,#85121,#85122,#85123,#85124,#85125,#85126,#85127,#85128,#85129,#85130,
#85131,#85132,#85133,#85134,#85135,#85136,#85137,#85138,#85139,#85140,#85141,
#85142,#85143,#85144,#85145,#85146,#85147,#85148,#85149,#85150,#85151,#85152,
#85153,#85154,#85155,#85156,#85157,#85158,#85159,#85160,#85161,#85162,#85163,
#85164,#85165,#85166,#85167,#85168,#85169,#85170,#85171,#85172,#85173,#85174,
#85175,#85176,#85177,#85178,#85179,#85180,#85181,#85182,#85183,#85184,#85185,
#85186,#85187,#85188,#85189,#85190,#85191,#85192,#85193,#85194,#85195,#85196,
#85197,#85198,#85199,#85200,#85201,#85202,#85203,#85204,#85205,#85206,#85207,
#85208,#85209,#85210,#85211,#85212,#85213,#85214,#85215,#85216,#85217,#85218,
#85219,#85220,#85221,#85222,#85223,#85224,#85225,#85226,#85227,#85228,#85229,
#85230,#85231,#85232,#85233,#85234,#85235,#85236,#85237,#85238,#85239,#85240,
#85241,#85242,#85243,#85244,#85245,#85246,#85247,#85248,#85249,#85250,#85251,
#85252,#85253,#85254,#85255,#85256,#85257,#85258,#85259,#85260,#85261,#85262,
#85263,#85264,#85265,#85266,#85267,#85268,#85269,#85270,#85271,#85272,#85273,
#85274,#85275,#85276,#85277,#85278,#85279,#85280,#85281,#85282,#85283,#85284,
#85285,#85286,#85287,#85288,#85289,#85290,#85291,#85292,#85293,#85294,#85295,
#85296,#85297,#85298,#85299,#85300,#85301,#85302,#85303,#85304,#85305,#85306,
#85307,#85308,#85309,#85310,#85311,#85312,#85313,#85314,#85315,#85316,#85317,
#85318,#85319,#85320,#85321,#85322,#85323,#85324,#85325,#85326,#85327,#85328),
 .UNSPECIFIED.,.F.,.F.,(4,2,2,2,2,2,2,2,2,2,2,2,2,2,2,2,2,2,2,2,2,2,2,2,
2,2,2,2,2,2,2,2,2,2,2,2,2,2,2,2,2,2,2,2,2,2,2,2,2,2,2,2,2,2,2,2,2,2,2,2,
2,2,2,2,2,2,2,2,2,2,2,2,2,2,2,2,2,2,2,2,2,2,2,2,2,2,2,2,2,2,2,2,2,2,2,2,
2,2,2,2,2,2,2,2,2,2,2,2,2,2,2,2,2,2,2,2,2,4),(-1.40860718540471,-1.39545808993048,
-1.38405624528616,-1.38177793059313,-1.3805200509377,-1.37944853194231,
-1.37810193303849,-1.37548652011566,-1.35956495703151,-1.35506264588485,
-1.33449830662054,-1.28614136850048,-1.2789919571089,-1.27608255110672,
-1.27428145157858,-1.27232580019934,-1.26965318149743,-1.26343338839415,
-1.23649954831244,-1.19597179011588,-1.17297882026764,-1.17012328492731,
-1.16874592682677,-1.1676719609531,-1.16643617728359,-1.16425891186825,
-1.15447735403195,-1.10554601526657,-1.07041727374431,-1.06612126926768,
-1.063579569456,-1.06163851526854,-1.05956481891129,-1.05631557804374,-1.04600323997315,
-1.0294397184734,-0.99657573807322,-0.982832105893307,-0.97598240220263,
-0.975672104818647,-0.970158116277952,-0.960090031442436,-0.958006977478143,
-0.956669998370231,-0.955599167368023,-0.954333955366218,-0.952021328308135,
-0.93999299257142,-0.888103875649836,-0.858245896180985,-0.854050891734989,
-0.851538739815541,-0.849602590843724,-0.847516780118267,-0.844211760805237,
-0.833400814558471,-0.815717905738926,-0.765188925544749,-0.748664645534886,
-0.746024308779368,-0.744672487254501,-0.743600790811616,-0.742347304807065,
-0.740088573175662,-0.729020101582865,-0.704034607495391,-0.649565231152326,
-0.64279328250916,-0.639946816886022,-0.638157450646532,-0.636192587999127,
-0.633467098953572,-0.626933960763457,-0.597388862372985,-0.557146604210194,
-0.552471553511539,-0.536616903204568,-0.534004059815459,-0.532658204128811,
-0.53158697035396,-0.530329075783386,-0.528049832044696,-0.516625192277147,
-0.490252175671931,-0.437797642683444,-0.430864864546959,-0.427991956806278,
-0.42619788771247,-0.424237438622548,-0.421535644843532,-0.415142795035289,
-0.368523243439547,-0.32763686859989,-0.322943240982788,-0.321206137539336,
-0.320181434593666,-0.319088610059422,-0.317575470945896,-0.313976333882245,
-0.276223914328954,-0.225951975819304,-0.218893242814937,-0.216053511747662,
-0.214086005908784,-0.212152793090381,-0.210202190533758,-0.205221672264368,
-0.167218897660105,-0.126530071387855,-0.112454765384175,-0.110146844098719,
-0.108756903288708,-0.107679218613484,-0.1064661349924,-0.104390619277934,
-0.0959745790071875,-0.0797771645789183,-0.0749587606043023),
 .UNSPECIFIED.);
#872=B_SPLINE_CURVE_WITH_KNOTS('',3,(#85330,#85331,#85332,#85333,#85334,
#85335,#85336,#85337,#85338,#85339,#85340,#85341,#85342,#85343,#85344,#85345,
#85346,#85347,#85348,#85349,#85350,#85351,#85352,#85353,#85354,#85355,#85356,
#85357,#85358,#85359,#85360,#85361,#85362,#85363,#85364,#85365,#85366,#85367,
#85368,#85369,#85370,#85371,#85372,#85373,#85374,#85375,#85376,#85377,#85378,
#85379,#85380,#85381,#85382,#85383,#85384,#85385,#85386,#85387,#85388,#85389,
#85390,#85391,#85392,#85393,#85394,#85395,#85396,#85397,#85398,#85399,#85400,
#85401,#85402,#85403,#85404,#85405,#85406,#85407,#85408,#85409,#85410,#85411,
#85412,#85413,#85414,#85415,#85416,#85417,#85418,#85419,#85420,#85421,#85422,
#85423,#85424,#85425,#85426,#85427,#85428,#85429,#85430,#85431,#85432,#85433,
#85434,#85435,#85436,#85437,#85438,#85439,#85440,#85441,#85442,#85443,#85444,
#85445,#85446,#85447,#85448,#85449,#85450,#85451,#85452,#85453,#85454,#85455,
#85456,#85457,#85458,#85459,#85460,#85461,#85462,#85463,#85464,#85465,#85466,
#85467,#85468,#85469,#85470,#85471,#85472,#85473,#85474,#85475,#85476,#85477,
#85478,#85479,#85480,#85481,#85482,#85483,#85484,#85485,#85486,#85487,#85488,
#85489,#85490,#85491,#85492,#85493,#85494,#85495,#85496,#85497,#85498,#85499,
#85500,#85501,#85502,#85503,#85504,#85505,#85506,#85507),.UNSPECIFIED.,
 .F.,.F.,(4,3,3,3,3,3,3,3,3,3,3,3,3,3,3,3,3,3,3,3,3,3,3,3,3,3,3,3,3,3,3,
3,3,3,3,3,3,3,3,3,3,3,3,3,3,3,3,3,3,3,3,3,3,3,3,3,3,3,3,4),(-66.322858757962,
-66.2209269068389,-66.1189508263109,-66.0167874108514,-65.9232056974837,
-65.8198109604357,-65.7165696783206,-65.6134497129282,-65.5103951447193,
-65.4073719363614,-65.3043460936888,-65.2012133269107,-65.0980242355009,
-64.9946522421192,-64.9243692475218,-64.820974510474,-64.7177332283587,
-64.6146132629665,-64.5115586947577,-64.4085354864001,-64.3055096437274,
-64.2023768769493,-64.0991877855396,-63.995815792158,-63.92553279756,-63.8221380605121,
-63.718896778397,-63.6157768130047,-63.5127222447958,-63.4096990364381,
-63.3066731937655,-63.2035404269875,-63.1003513355777,-62.9969793421961,
-62.9266963475981,-62.8233016105501,-62.7200603284353,-62.6169403630429,
-62.513885794834,-62.4108625864763,-62.3078367438037,-62.2047039770256,
-62.1015148856157,-61.998142892234,-61.9278598976362,-61.8244651605883,
-61.7212238784734,-61.6181039130811,-61.5150493448724,-61.4120261365148,
-61.3090002938418,-61.2058675270639,-61.1026784356542,-60.9993064422726,
-60.9290234476744,-60.8220651862382,-60.7139755891884,-60.6074364851714,
-60.4985716416052,-60.3897067980389),.UNSPECIFIED.);
#873=B_SPLINE_CURVE_WITH_KNOTS('',3,(#85508,#85509,#85510,#85511),
 .UNSPECIFIED.,.F.,.F.,(4,4),(-60.3897037700498,-60.0402339961103),
 .UNSPECIFIED.);
#874=B_SPLINE_CURVE_WITH_KNOTS('',3,(#85517,#85518,#85519,#85520,#85521,
#85522),.UNSPECIFIED.,.F.,.F.,(4,2,4),(-0.0750400054689081,-0.0533928212318036,
-0.000629601363601487),.UNSPECIFIED.);
#875=B_SPLINE_CURVE_WITH_KNOTS('',3,(#85523,#85524,#85525,#85526,#85527,
#85528,#85529,#85530,#85531,#85532,#85533,#85534,#85535,#85536,#85537,#85538,
#85539,#85540,#85541,#85542,#85543,#85544,#85545,#85546,#85547,#85548,#85549,
#85550,#85551,#85552,#85553,#85554,#85555,#85556,#85557,#85558,#85559,#85560,
#85561,#85562,#85563,#85564,#85565,#85566,#85567,#85568,#85569,#85570,#85571,
#85572,#85573,#85574,#85575,#85576,#85577,#85578,#85579,#85580,#85581,#85582,
#85583,#85584,#85585,#85586,#85587,#85588,#85589,#85590,#85591,#85592,#85593,
#85594,#85595,#85596,#85597,#85598,#85599,#85600,#85601,#85602,#85603,#85604,
#85605,#85606,#85607,#85608,#85609,#85610,#85611,#85612,#85613,#85614,#85615,
#85616,#85617,#85618,#85619,#85620,#85621,#85622,#85623,#85624,#85625,#85626,
#85627,#85628,#85629,#85630,#85631,#85632,#85633,#85634,#85635,#85636,#85637,
#85638,#85639,#85640,#85641,#85642,#85643,#85644,#85645,#85646,#85647,#85648,
#85649,#85650,#85651,#85652,#85653,#85654,#85655,#85656,#85657,#85658,#85659,
#85660,#85661,#85662,#85663,#85664,#85665,#85666,#85667,#85668,#85669,#85670,
#85671,#85672,#85673,#85674,#85675,#85676,#85677,#85678,#85679,#85680,#85681,
#85682,#85683,#85684,#85685,#85686,#85687,#85688,#85689,#85690,#85691,#85692,
#85693,#85694,#85695,#85696,#85697,#85698,#85699,#85700,#85701,#85702,#85703,
#85704,#85705,#85706,#85707,#85708,#85709,#85710,#85711,#85712,#85713,#85714,
#85715,#85716,#85717,#85718,#85719,#85720,#85721,#85722,#85723,#85724,#85725,
#85726,#85727,#85728,#85729,#85730,#85731,#85732,#85733,#85734,#85735,#85736,
#85737,#85738,#85739,#85740,#85741,#85742,#85743,#85744,#85745,#85746,#85747,
#85748,#85749,#85750,#85751,#85752,#85753,#85754,#85755,#85756,#85757,#85758,
#85759,#85760,#85761,#85762,#85763,#85764,#85765,#85766,#85767,#85768,#85769,
#85770,#85771,#85772,#85773,#85774),.UNSPECIFIED.,.F.,.F.,(4,2,2,2,2,2,
2,2,2,2,2,2,2,2,2,2,2,2,2,2,2,2,2,2,2,2,2,2,2,2,2,2,2,2,2,2,2,2,2,2,2,2,
2,2,2,2,2,2,2,2,2,2,2,2,2,2,2,2,2,2,2,2,2,2,2,2,2,2,2,2,2,2,2,2,2,2,2,2,
2,2,2,2,2,2,2,2,2,2,2,2,2,2,2,2,2,2,2,2,2,2,2,2,2,2,2,2,2,2,2,2,2,2,2,2,
2,2,2,2,2,2,2,2,2,2,2,4),(-2.66809500613749,-2.66003737079873,-2.65567972419421,
-2.65426658705818,-2.65319922550382,-2.65216891022884,-2.65098887662144,
-2.64906346401233,-2.64299730418109,-2.64171516263787,-2.63391396391436,
-2.58086173899162,-2.56301613163371,-2.55213395024574,-2.54882039643755,
-2.54673224354217,-2.54479601378358,-2.54228671783658,-2.53810299894828,
-2.50874889582129,-2.46751320115535,-2.452047531728,-2.44662577265192,-2.44402429013868,
-2.44191582684355,-2.44070265038365,-2.44069954126522,-2.44069641315407,
-2.44069326608247,-2.44069009995937,-2.44068691443319,-2.44068370945783,
-2.44068048479903,-2.44067724042621,-2.44067397628221,-2.44067069219663,
-2.44066738796819,-2.44066406353025,-2.44066073156736,-2.44065738525505,
-2.44065401781087,-2.44065062905198,-2.44064720769557,-2.43961927545029,
-2.43823982570499,-2.4353731301731,-2.39981442473688,-2.36690462497572,
-2.344124633947,-2.33844102161752,-2.3358640429016,-2.33392451108213,-2.33209915097093,
-2.3295628695129,-2.32295878519058,-2.26677128155561,-2.24294981956697,
-2.23219106010818,-2.22995079072762,-2.22870125010139,-2.22762904750754,
-2.22627160190742,-2.22412178656339,-2.21301973096917,-2.16174691742912,
-2.13313406475128,-2.12671135454216,-2.1240042704081,-2.122042650224,-2.12024935039312,
-2.11738167453837,-2.11048217807699,-2.05758353202986,-2.03154305390505,
-2.02020117751967,-2.01792645294227,-2.01666943047337,-2.01559795954986,
-2.0142505530444,-2.01163102257304,-1.99562806976032,-1.9901364525329,-1.97569906836753,
-1.94280344370365,-1.92623589621873,-1.91592271366936,-1.91267332660119,
-1.91059957214408,-1.90865848884485,-1.90611678859568,-1.9018208999285,
-1.8666880603306,-1.81772896417468,-1.80801166462807,-1.80583884657001,
-1.80460405019258,-1.80352996207818,-1.80215115513934,-1.79928817885767,
-1.7632764622433,-1.73051723134771,-1.7079751678773,-1.70232341243381,-1.69975212318208,
-1.69781331258464,-1.69598601545781,-1.69344284687175,-1.68679602284043,
-1.63101292099283,-1.59811451212367,-1.59456756021743,-1.59306309617033,
-1.59197154165544,-1.59094404025414,-1.58919363814061,-1.58441434265556,
-1.54724248996085,-1.49696430469026,-1.49056164232697,-1.48785778282483,
-1.48589659592665,-1.48410238033114,-1.48123037997351,-1.47430567066695,
-1.42173351548525,-1.40860718540471),.UNSPECIFIED.);
#876=B_SPLINE_CURVE_WITH_KNOTS('',3,(#85776,#85777,#85778,#85779,#85780,
#85781,#85782,#85783,#85784,#85785),.UNSPECIFIED.,.F.,.F.,(4,1,1,1,1,1,
1,4),(-60.0402339961103,-59.9301869977125,-58.9313505477506,-57.9325140977887,
-56.9336776478269,-55.934841197865,-54.9360047479031,-54.1065275196808),
 .UNSPECIFIED.);
#877=B_SPLINE_CURVE_WITH_KNOTS('',3,(#85786,#85787,#85788,#85789,#85790,
#85791,#85792,#85793,#85794,#85795,#85796,#85797,#85798,#85799,#85800,#85801,
#85802,#85803,#85804,#85805,#85806,#85807),.UNSPECIFIED.,.F.,.F.,(4,2,2,
2,2,2,2,2,2,2,4),(-2.66746648764681,-2.64323635106775,-2.63610435627689,
-2.63431343163605,-2.63309845601206,-2.63208936873757,-2.63101477987198,
-2.62962873109103,-2.62672769851142,-2.59980703035293,-2.59336498099373),
 .UNSPECIFIED.);
#878=B_SPLINE_CURVE_WITH_KNOTS('',3,(#85812,#85813,#85814,#85815,#85816,
#85817,#85818,#85819,#85820,#85821,#85822,#85823,#85824,#85825,#85826,#85827,
#85828,#85829,#85830,#85831,#85832,#85833,#85834,#85835,#85836,#85837,#85838,
#85839,#85840,#85841,#85842,#85843,#85844,#85845,#85846,#85847,#85848,#85849,
#85850,#85851,#85852,#85853,#85854,#85855,#85856,#85857,#85858,#85859,#85860,
#85861,#85862,#85863,#85864,#85865,#85866,#85867,#85868,#85869,#85870,#85871,
#85872,#85873,#85874,#85875,#85876,#85877,#85878,#85879,#85880,#85881,#85882,
#85883,#85884,#85885,#85886,#85887,#85888,#85889,#85890,#85891,#85892,#85893,
#85894,#85895,#85896,#85897,#85898,#85899,#85900,#85901,#85902,#85903,#85904,
#85905,#85906,#85907,#85908,#85909,#85910,#85911,#85912,#85913,#85914,#85915,
#85916,#85917,#85918,#85919,#85920,#85921,#85922,#85923,#85924,#85925,#85926,
#85927,#85928,#85929,#85930,#85931,#85932,#85933,#85934,#85935,#85936,#85937,
#85938,#85939,#85940,#85941,#85942,#85943,#85944,#85945,#85946,#85947,#85948,
#85949,#85950,#85951,#85952,#85953,#85954,#85955,#85956,#85957,#85958,#85959,
#85960,#85961,#85962,#85963,#85964,#85965,#85966,#85967,#85968,#85969,#85970,
#85971,#85972,#85973,#85974,#85975,#85976,#85977,#85978,#85979,#85980,#85981,
#85982,#85983,#85984,#85985,#85986,#85987,#85988,#85989,#85990,#85991,#85992,
#85993,#85994,#85995,#85996,#85997,#85998,#85999,#86000,#86001,#86002,#86003,
#86004,#86005,#86006,#86007,#86008,#86009,#86010,#86011,#86012,#86013,#86014,
#86015,#86016,#86017,#86018,#86019,#86020,#86021,#86022,#86023,#86024,#86025,
#86026,#86027,#86028,#86029,#86030,#86031,#86032,#86033,#86034,#86035,#86036,
#86037,#86038,#86039,#86040,#86041,#86042,#86043,#86044,#86045,#86046,#86047,
#86048,#86049,#86050,#86051,#86052,#86053),.UNSPECIFIED.,.F.,.F.,(4,2,2,
2,2,2,2,2,2,2,2,2,2,2,2,2,2,2,2,2,2,2,2,2,2,2,2,2,2,2,2,2,2,2,2,2,2,2,2,
2,2,2,2,2,2,2,2,2,2,2,2,2,2,2,2,2,2,2,2,2,2,2,2,2,2,2,2,2,2,2,2,2,2,2,2,
2,2,2,2,2,2,2,2,2,2,2,2,2,2,2,2,2,2,2,2,2,2,2,2,2,2,2,2,2,2,2,2,2,2,2,2,
2,2,2,2,2,2,2,2,2,4),(-1.40838688772306,-1.38230244357366,-1.3689629544219,
-1.36540809648996,-1.3632670538202,-1.3613458718201,-1.35890266866713,-1.3550283155242,
-1.33395525283396,-1.27614236927097,-1.26118233595888,-1.2588344111419,
-1.25743266749409,-1.2563533252078,-1.2551467114111,-1.25310066828271,-1.24504355176718,
-1.22986487393631,-1.18997000193031,-1.1589272040029,-1.15470580671402,
-1.15218595694187,-1.15024860976343,-1.14816616428751,-1.14487637778995,
-1.13420309883885,-1.11683233307578,-1.06813033440054,-1.06161521720435,
-1.04899334516723,-1.04675771195742,-1.04537434325928,-1.04429995546135,
-1.04306848022654,-1.04091018720103,-1.03139827240251,-0.982246778625874,
-0.947052503044537,-0.94275632244464,-0.940214801714153,-0.938274047406892,
-0.936200829559232,-0.932952668602648,-0.922646540217495,-0.906095637795037,
-0.873245520663565,-0.860327841072428,-0.837625961972406,-0.834772518271112,
-0.833395802704332,-0.832322165531018,-0.831086565469334,-0.828909157661812,
-0.819119234990314,-0.770211171374527,-0.735095479701707,-0.730800735191928,
-0.728259768505998,-0.72631926709606,-0.724246154408423,-0.720997813714003,
-0.710688211446137,-0.694128968940473,-0.661273965145536,-0.647500265802612,
-0.640732865430314,-0.639125212782759,-0.625206095140421,-0.622905976907174,
-0.62151840927512,-0.620441125137846,-0.61922687568498,-0.617145737159202,
-0.608657739676505,-0.59225104333614,-0.550125200292749,-0.522888990514207,
-0.518762151511242,-0.516270269944921,-0.514337569265241,-0.512243345501892,
-0.508898821763093,-0.497717993373553,-0.479181723901062,-0.434933754979829,
-0.413700363030104,-0.410884809280078,-0.409515665871969,-0.408442841512717,
-0.407202392723714,-0.40500245852627,-0.394872764219282,-0.373279481527361,
-0.365786413232853,-0.314761438692117,-0.307738844509065,-0.304851387375707,
-0.303054887736032,-0.301097089088425,-0.298408602847309,-0.292092278485095,
-0.264359179113338,-0.222328372943981,-0.201736020462186,-0.198933982706451,
-0.197567544224861,-0.196546512687276,-0.195348174400184,-0.193343619419814,
-0.190871317984728,-0.185820315614274,-0.171894974603336,-0.15129838099146,
-0.103002734319542,-0.0958553337604737,-0.092947074412366,-0.0911467847291241,
-0.0891920915881641,-0.0865209243899677,-0.0803051558083365,-0.0750400054689081),
 .UNSPECIFIED.);
#879=B_SPLINE_CURVE_WITH_KNOTS('',3,(#86054,#86055,#86056,#86057,#86058,
#86059,#86060,#86061,#86062,#86063,#86064,#86065,#86066,#86067,#86068,#86069,
#86070,#86071,#86072,#86073,#86074,#86075,#86076,#86077,#86078,#86079,#86080,
#86081,#86082,#86083,#86084,#86085,#86086,#86087,#86088,#86089,#86090,#86091,
#86092,#86093,#86094,#86095,#86096,#86097,#86098,#86099,#86100,#86101,#86102,
#86103,#86104,#86105,#86106,#86107,#86108,#86109,#86110,#86111,#86112,#86113,
#86114,#86115,#86116,#86117,#86118,#86119,#86120,#86121,#86122,#86123,#86124,
#86125,#86126,#86127,#86128,#86129,#86130,#86131,#86132,#86133,#86134,#86135,
#86136,#86137,#86138,#86139,#86140,#86141,#86142,#86143,#86144,#86145,#86146,
#86147,#86148,#86149,#86150,#86151,#86152,#86153,#86154,#86155,#86156,#86157,
#86158,#86159,#86160,#86161,#86162,#86163,#86164,#86165,#86166,#86167,#86168,
#86169,#86170,#86171,#86172,#86173,#86174,#86175,#86176,#86177,#86178,#86179,
#86180,#86181,#86182,#86183,#86184,#86185,#86186,#86187,#86188,#86189,#86190,
#86191,#86192,#86193,#86194,#86195,#86196,#86197,#86198,#86199,#86200,#86201,
#86202,#86203,#86204,#86205,#86206,#86207,#86208,#86209,#86210,#86211,#86212,
#86213,#86214,#86215,#86216,#86217,#86218,#86219,#86220,#86221,#86222,#86223,
#86224,#86225,#86226,#86227,#86228,#86229,#86230,#86231,#86232,#86233,#86234,
#86235,#86236,#86237,#86238,#86239,#86240,#86241,#86242,#86243,#86244,#86245,
#86246,#86247,#86248,#86249,#86250,#86251,#86252,#86253,#86254,#86255,#86256,
#86257,#86258,#86259,#86260,#86261,#86262,#86263,#86264,#86265,#86266,#86267,
#86268,#86269,#86270,#86271,#86272,#86273,#86274,#86275,#86276,#86277,#86278,
#86279,#86280,#86281,#86282,#86283,#86284,#86285),.UNSPECIFIED.,.F.,.F.,
(4,2,2,2,2,2,2,2,2,2,2,2,2,2,2,2,2,2,2,2,2,2,2,2,2,2,2,2,2,2,2,2,2,2,2,
2,2,2,2,2,2,2,2,2,2,2,2,2,2,2,2,2,2,2,2,2,2,2,2,2,2,2,2,2,2,2,2,2,2,2,2,
2,2,2,2,2,2,2,2,2,2,2,2,2,2,2,2,2,2,2,2,2,2,2,2,2,2,2,2,2,2,2,2,2,2,2,2,
2,2,2,2,2,2,2,2,4),(-2.59336498099373,-2.58612377715144,-2.57460295655263,
-2.54602644095796,-2.53212826401375,-2.52852472099612,-2.52637284115968,
-2.52445355466388,-2.52202850292267,-2.51729671326334,-2.47985852346038,
-2.42950698100758,-2.4230330905425,-2.42114165560786,-2.42013068020849,
-2.41905739996276,-2.41768570023441,-2.41548870872608,-2.40365158526575,
-2.34625429950801,-2.32969062991946,-2.31937983627995,-2.31613118864746,
-2.3140579029223,-2.31211725613926,-2.30957612426245,-2.30528118904737,
-2.2701552012624,-2.2212038755009,-2.21149260018589,-2.20932053545729,-2.20808607523894,
-2.20701222055165,-2.20563363609001,-2.2027708554975,-2.16714451094693,
-2.13426170118579,-2.11770520689291,-2.10739755892156,-2.10414919953203,
-2.10207592884624,-2.10013517747864,-2.09759373743708,-2.09329789758949,
-2.05811272113606,-2.00897230617553,-1.99947907606189,-1.99732216214529,
-1.99609100999797,-1.99501660919084,-1.9936328259664,-1.99139573413456,
-1.9787459135555,-1.97653424229513,-1.97434496400237,-1.92392173045384,
-1.90628615561207,-1.89549731307634,-1.89219485829476,-1.89010970551398,
-1.88817350573697,-1.88566035165332,-1.88146164769916,-1.85141490721498,
-1.79974588301394,-1.78774089675046,-1.78542972168894,-1.78416490230857,
-1.78309416754148,-1.7817570060096,-1.77967310600665,-1.76959088583284,
-1.76408849451663,-1.75666055670907,-1.74315355697832,-1.71027191066444,
-1.69371826756403,-1.68341173156511,-1.68016336965071,-1.67809001251601,
-1.67614912062268,-1.67360741055167,-1.66931092146314,-1.6340939351491,
-1.5848491215704,-1.57547147075961,-1.57332268396228,-1.57209327523349,
-1.57101851553897,-1.56963179330887,-1.56738508325563,-1.55455222370681,
-1.55238617999346,-1.50510585335559,-1.47658175093414,-1.47016979631437,
-1.46746461537597,-1.46550341737666,-1.46370984438008,-1.46084029569995,
-1.45392885652446,-1.40119783292654,-1.37504354039233,-1.36367304688529,
-1.36139677139001,-1.36013945244606,-1.35906806863937,-1.35772120402661,
-1.3551039967121,-1.33914203000199,-1.33419803675157,-1.32855203675639,
-1.28159297975054,-1.28014689813355,-1.26110770786606,-1.25972990448764),
 .UNSPECIFIED.);
#880=B_SPLINE_CURVE_WITH_KNOTS('',3,(#86291,#86292,#86293,#86294,#86295,
#86296,#86297,#86298,#86299,#86300,#86301,#86302,#86303,#86304,#86305,#86306),
 .UNSPECIFIED.,.F.,.F.,(4,2,2,2,2,2,2,4),(-0.0747633067458267,-0.0741278680970252,
-0.0730557645895703,-0.0718087286992157,-0.0695788634709163,-0.0589815407426049,
-0.0357413577562223,-0.00062954340747806),.UNSPECIFIED.);
#881=B_SPLINE_CURVE_WITH_KNOTS('',3,(#86307,#86308,#86309,#86310,#86311,
#86312,#86313,#86314,#86315,#86316,#86317,#86318,#86319,#86320,#86321,#86322,
#86323,#86324,#86325,#86326,#86327,#86328,#86329,#86330,#86331,#86332,#86333,
#86334,#86335,#86336,#86337,#86338,#86339,#86340,#86341,#86342,#86343,#86344,
#86345,#86346,#86347,#86348,#86349,#86350,#86351,#86352,#86353,#86354,#86355,
#86356,#86357,#86358,#86359,#86360,#86361,#86362,#86363,#86364,#86365,#86366,
#86367,#86368,#86369,#86370,#86371,#86372,#86373,#86374,#86375,#86376,#86377,
#86378,#86379,#86380,#86381,#86382,#86383,#86384,#86385,#86386,#86387,#86388,
#86389,#86390,#86391,#86392,#86393,#86394,#86395,#86396,#86397,#86398,#86399,
#86400,#86401,#86402,#86403,#86404,#86405,#86406,#86407,#86408,#86409,#86410,
#86411,#86412,#86413,#86414,#86415,#86416,#86417,#86418,#86419,#86420,#86421,
#86422,#86423,#86424,#86425,#86426,#86427,#86428,#86429,#86430,#86431,#86432,
#86433,#86434,#86435,#86436,#86437,#86438,#86439,#86440,#86441,#86442,#86443,
#86444,#86445,#86446,#86447,#86448,#86449,#86450,#86451,#86452,#86453,#86454,
#86455,#86456,#86457,#86458,#86459,#86460,#86461,#86462,#86463,#86464,#86465,
#86466,#86467,#86468,#86469,#86470,#86471,#86472,#86473,#86474,#86475,#86476,
#86477,#86478,#86479,#86480,#86481,#86482,#86483,#86484,#86485,#86486,#86487,
#86488,#86489,#86490,#86491,#86492,#86493,#86494,#86495,#86496,#86497,#86498,
#86499,#86500,#86501,#86502,#86503,#86504,#86505,#86506,#86507,#86508,#86509,
#86510,#86511,#86512,#86513,#86514,#86515,#86516,#86517,#86518,#86519,#86520,
#86521,#86522,#86523,#86524,#86525,#86526,#86527,#86528,#86529,#86530,#86531,
#86532,#86533,#86534,#86535,#86536,#86537,#86538,#86539,#86540,#86541,#86542,
#86543,#86544,#86545,#86546,#86547,#86548,#86549,#86550,#86551,#86552,#86553,
#86554,#86555,#86556,#86557,#86558,#86559,#86560,#86561,#86562,#86563,#86564,
#86565,#86566,#86567,#86568,#86569,#86570,#86571,#86572,#86573,#86574),
 .UNSPECIFIED.,.F.,.F.,(4,2,2,2,2,2,2,2,2,2,2,2,2,2,2,2,2,2,2,2,2,2,2,2,
2,2,2,2,2,2,2,2,2,2,2,2,2,2,2,2,2,2,2,2,2,2,2,2,2,2,2,2,2,2,2,2,2,2,2,2,
2,2,2,2,2,2,2,2,2,2,2,2,2,2,2,2,2,2,2,2,2,2,2,2,2,2,2,2,2,2,2,2,2,2,2,2,
2,2,2,2,2,2,2,2,2,2,2,2,2,2,2,2,2,2,2,2,2,2,2,2,2,2,2,2,2,2,2,2,2,2,2,2,
2,4),(-2.66773872145495,-2.64241252558027,-2.63928554969506,-2.63713947602669,
-2.63533867351105,-2.63342472947524,-2.63105557271983,-2.62742202621152,
-2.61031671120093,-2.59812617594819,-2.55348115611806,-2.53501219789282,
-2.53117993176174,-2.52962817609444,-2.52852850087925,-2.52751377117936,
-2.5258273549798,-2.52146094153608,-2.47375191666192,-2.44446095946491,
-2.43444799925098,-2.42965975435597,-2.42576618372853,-2.42356262739359,
-2.42354995819552,-2.4235368515971,-2.42352329137586,-2.42350926072277,
-2.42349473912475,-2.42347970994217,-2.42346415578335,-2.4234480568527,
-2.42343139254774,-2.42341414145426,-2.42339628125805,-2.42337778868366,
-2.4233586395713,-2.42333880874003,-2.42331826995378,-2.42329699594181,
-2.42327495825973,-2.42325212674527,-2.42323282571979,-2.42321027756231,
-2.42318393277581,-2.42315314833329,-2.42311717188563,-2.42307512336121,
-2.42302736684747,-2.42108673959665,-2.41854502817043,-2.41424775666325,
-2.37918547353218,-2.33040402256907,-2.32049585296989,-2.31831050487343,
-2.31707318244614,-2.31599982764569,-2.31462578450445,-2.3124207068573,
-2.30036184922826,-2.24416348853271,-2.22062564956556,-2.21484159161938,
-2.21224675635151,-2.21030485039764,-2.20848530346745,-2.20596988674875,
-2.1994925453796,-2.14221577091108,-2.11910848208663,-2.10854717635702,
-2.10631954953316,-2.10507298661917,-2.10400080970302,-2.10264013901542,
-2.0999577347487,-2.08228655993597,-2.033887122098,-2.00890354709408,-2.0029308528024,
-2.00030214126094,-1.99835463635392,-1.99654399145709,-1.99406302454134,
-1.98779240179784,-1.92885811313851,-1.90677667843905,-1.89650476019713,
-1.89429543948097,-1.89305285336334,-1.89198016977548,-1.89061377415086,
-1.88843395598268,-1.87682215435673,-1.87294119289219,-1.87270452445276,
-1.8658392028681,-1.85210677914542,-1.81922599238434,-1.80267118267403,
-1.79236438822734,-1.78911619381477,-1.78704300342312,-1.78510230965067,
-1.78256091967883,-1.77826510762717,-1.74307236981169,-1.69390412678815,
-1.68444508453741,-1.68229063846524,-1.68106005453799,-1.6799856052173,
-1.67860104349444,-1.67570770147822,-1.64967487965741,-1.6115097133864,
-1.58248330931025,-1.578087932836,-1.57576448500794,-1.57385298149189,-1.57162897726566,
-1.56780092678016,-1.55274039453732,-1.50057476592015,-1.48173019249633,
-1.47243485082074,-1.47029206737946,-1.46906402334406,-1.46798910731072,
-1.466600402696,-1.46368594057752,-1.43364138024875,-1.40838688772306),
 .UNSPECIFIED.);
#882=B_SPLINE_CURVE_WITH_KNOTS('',3,(#86576,#86577,#86578,#86579,#86580,
#86581,#86582,#86583,#86584,#86585,#86586,#86587,#86588,#86589,#86590,#86591,
#86592,#86593,#86594,#86595,#86596,#86597,#86598,#86599,#86600,#86601,#86602,
#86603,#86604,#86605,#86606,#86607,#86608,#86609,#86610,#86611,#86612,#86613,
#86614,#86615,#86616,#86617,#86618,#86619,#86620,#86621,#86622,#86623,#86624,
#86625,#86626,#86627,#86628,#86629,#86630,#86631,#86632,#86633,#86634,#86635,
#86636,#86637,#86638,#86639,#86640,#86641,#86642,#86643,#86644,#86645,#86646,
#86647,#86648,#86649,#86650,#86651,#86652,#86653,#86654,#86655,#86656,#86657,
#86658,#86659,#86660,#86661,#86662,#86663,#86664,#86665,#86666,#86667,#86668,
#86669,#86670,#86671,#86672,#86673,#86674,#86675,#86676,#86677,#86678,#86679,
#86680,#86681,#86682,#86683,#86684,#86685,#86686,#86687,#86688,#86689,#86690,
#86691,#86692,#86693,#86694,#86695,#86696,#86697,#86698,#86699,#86700,#86701,
#86702,#86703,#86704,#86705,#86706,#86707,#86708,#86709,#86710,#86711,#86712,
#86713,#86714,#86715,#86716,#86717,#86718,#86719,#86720,#86721,#86722,#86723,
#86724,#86725,#86726,#86727,#86728,#86729,#86730,#86731,#86732,#86733,#86734,
#86735,#86736,#86737,#86738,#86739,#86740,#86741,#86742,#86743,#86744,#86745,
#86746,#86747,#86748,#86749,#86750,#86751,#86752,#86753,#86754,#86755,#86756,
#86757,#86758,#86759,#86760,#86761,#86762,#86763,#86764,#86765,#86766,#86767,
#86768,#86769,#86770,#86771,#86772,#86773,#86774,#86775,#86776,#86777,#86778,
#86779,#86780,#86781,#86782,#86783,#86784,#86785,#86786,#86787,#86788,#86789,
#86790,#86791,#86792,#86793),.UNSPECIFIED.,.F.,.F.,(4,2,2,2,2,2,2,2,2,2,
2,2,2,2,2,2,2,2,2,2,2,2,2,2,2,2,2,2,2,2,2,2,2,2,2,2,2,2,2,2,2,2,2,2,2,2,
2,2,2,2,2,2,2,2,2,2,2,2,2,2,2,2,2,2,2,2,2,2,2,2,2,2,2,2,2,2,2,2,2,2,2,2,
2,2,2,2,2,2,2,2,2,2,2,2,2,2,2,2,2,2,2,2,2,2,2,2,2,2,4),(-1.25972990448764,
-1.25734657803934,-1.2549378371491,-1.25302008873775,-1.25085789112559,
-1.24720806171467,-1.23275541257723,-1.18236867555363,-1.15270122528572,
-1.14978674158883,-1.14839798039503,-1.14732299543195,-1.14609485382689,
-1.14395184167295,-1.13465490831496,-1.11580348097264,-1.07535035023734,
-1.06307169323884,-1.0484919271737,-1.04470596277304,-1.04249151506882,
-1.04057923218866,-1.03824355543878,-1.03379049295154,-1.00275461896363,
-0.95477787149643,-0.940188171153965,-0.937855789338092,-0.936458547161109,
-0.935379753962438,-0.934170502638011,-0.932112819458008,-0.923917714333937,
-0.908352379753073,-0.866771560268404,-0.854701250343117,-0.836944102576898,
-0.833267479208628,-0.830884677684527,-0.828969179144978,-0.826789683687461,
-0.823061780392079,-0.807615908699947,-0.75602335284784,-0.728679195530954,
-0.725774719653931,-0.724387870099407,-0.723313046637944,-0.722083613211083,
-0.719934882333577,-0.710559332764686,-0.661284102723659,-0.626051785632179,
-0.621754785433216,-0.619212915369639,-0.617271972336409,-0.615198628524614,
-0.611950428120897,-0.601645504903761,-0.58509780259168,-0.552248689487846,
-0.539755468425894,-0.516621377773021,-0.513763443981024,-0.512385776512252,
-0.511311967519572,-0.510076813766818,-0.507901732814191,-0.498147754683301,
-0.449204440910873,-0.414076862766473,-0.40978089006016,-0.407239455898081,
-0.405298746730069,-0.403225556779169,-0.399977397106138,-0.389670915418459,
-0.373119106130488,-0.340268621774019,-0.327240925826132,-0.31850684934553,
-0.304211592955686,-0.30189193036109,-0.300498556793765,-0.299420448437986,
-0.298209391337645,-0.296142923050037,-0.287837897838107,-0.271958943551731,
-0.225888947742334,-0.20163851679482,-0.197623479772591,-0.195164524654203,
-0.193294488448743,-0.19126637998537,-0.188075034363523,-0.184319691678446,
-0.177183092180901,-0.159610048660014,-0.109454259189925,-0.0924346847407807,
-0.0897757999029687,-0.0884201282119508,-0.0873483077285469,-0.0860980469878534,
-0.0838535675899181,-0.0730192674453548,-0.0489118854442952,-0.000629479492146207),
 .UNSPECIFIED.);
#883=B_SPLINE_CURVE_WITH_KNOTS('',3,(#86794,#86795,#86796,#86797,#86798,
#86799,#86800,#86801,#86802,#86803,#86804,#86805,#86806,#86807,#86808,#86809,
#86810,#86811,#86812,#86813,#86814,#86815),.UNSPECIFIED.,.F.,.F.,(4,2,2,
2,2,2,2,2,2,2,4),(-2.66777374952406,-2.65998003102873,-2.65468366447004,
-2.65224032161588,-2.6503584941431,-2.64851781255906,-2.64669143457867,
-2.64415107708231,-2.63895997732565,-2.62644993719922,-2.59336156192323),
 .UNSPECIFIED.);
#884=B_SPLINE_CURVE_WITH_KNOTS('',3,(#86820,#86821,#86822,#86823,#86824,
#86825,#86826,#86827,#86828,#86829,#86830,#86831,#86832,#86833,#86834,#86835,
#86836,#86837,#86838,#86839,#86840,#86841,#86842,#86843,#86844,#86845,#86846,
#86847,#86848,#86849,#86850,#86851,#86852,#86853,#86854,#86855,#86856,#86857,
#86858,#86859,#86860,#86861,#86862,#86863,#86864,#86865,#86866,#86867,#86868,
#86869,#86870,#86871,#86872,#86873,#86874,#86875,#86876,#86877,#86878,#86879,
#86880,#86881,#86882,#86883,#86884,#86885,#86886,#86887,#86888,#86889,#86890,
#86891,#86892,#86893,#86894,#86895,#86896,#86897,#86898,#86899,#86900,#86901,
#86902,#86903,#86904,#86905,#86906,#86907,#86908,#86909,#86910,#86911,#86912,
#86913,#86914,#86915,#86916,#86917,#86918,#86919,#86920,#86921,#86922,#86923,
#86924,#86925,#86926,#86927,#86928,#86929,#86930,#86931,#86932,#86933,#86934,
#86935,#86936,#86937,#86938,#86939,#86940,#86941,#86942,#86943,#86944,#86945,
#86946,#86947,#86948,#86949,#86950,#86951,#86952,#86953,#86954,#86955,#86956,
#86957,#86958,#86959,#86960,#86961,#86962,#86963,#86964,#86965,#86966,#86967,
#86968,#86969,#86970,#86971,#86972,#86973,#86974,#86975,#86976,#86977,#86978,
#86979,#86980,#86981,#86982,#86983,#86984,#86985,#86986,#86987,#86988,#86989,
#86990,#86991,#86992,#86993,#86994,#86995,#86996,#86997,#86998,#86999,#87000,
#87001,#87002,#87003,#87004,#87005,#87006,#87007,#87008,#87009,#87010,#87011,
#87012,#87013,#87014,#87015,#87016,#87017,#87018,#87019,#87020,#87021,#87022,
#87023,#87024,#87025,#87026,#87027,#87028,#87029,#87030,#87031,#87032,#87033,
#87034,#87035,#87036,#87037,#87038,#87039,#87040,#87041),.UNSPECIFIED.,
 .F.,.F.,(4,2,2,2,2,2,2,2,2,2,2,2,2,2,2,2,2,2,2,2,2,2,2,2,2,2,2,2,2,2,2,
2,2,2,2,2,2,2,2,2,2,2,2,2,2,2,2,2,2,2,2,2,2,2,2,2,2,2,2,2,2,2,2,2,2,2,2,
2,2,2,2,2,2,2,2,2,2,2,2,2,2,2,2,2,2,2,2,2,2,2,2,2,2,2,2,2,2,2,2,2,2,2,2,
2,2,2,2,2,2,2,4),(-1.4084593254711,-1.36760689910925,-1.35571434309166,
-1.35117925453299,-1.34787084561134,-1.34640836269805,-1.34532365970278,
-1.34413477147142,-1.34216882516782,-1.33576371835975,-1.33420781199927,
-1.31962127788188,-1.26057978066336,-1.24627009272878,-1.24250840802672,
-1.24029957652405,-1.2383869228092,-1.23604419783816,-1.23155727455813,
-1.19919559199268,-1.15901192704814,-1.15407997627054,-1.13813083897073,
-1.13551432467702,-1.13416761743711,-1.13309625339311,-1.13183884103811,
-1.12956208907755,-1.11818343024146,-1.09199414519246,-1.0392716360922,
-1.03235709909658,-1.02948706073595,-1.02769341606812,-1.02573233367823,
-1.0230276595747,-1.0166185298546,-0.988121510261783,-0.937199226502322,
-0.92570675954955,-0.923533677672336,-0.922169221180612,-0.921096560420311,
-0.919852296675333,-0.917635805323615,-0.907255903943466,-0.884795019387741,
-0.82642782159497,-0.820075908530418,-0.817581030184306,-0.815766627036285,
-0.813821099518584,-0.811205575278863,-0.805308102231652,-0.780912575796105,
-0.730249222676817,-0.714074343533306,-0.711447954441862,-0.710099173965592,
-0.709027740462902,-0.707772076114364,-0.705503132941652,-0.694258425547811,
-0.6685932424672,-0.615123230736673,-0.608267079429076,-0.605406761343438,
-0.603614966737304,-0.601652505505277,-0.598939683635388,-0.592481599269618,
-0.538617341485635,-0.50233491230343,-0.499482648454923,-0.498106108188645,
-0.497032422355204,-0.495796556867449,-0.493618179733451,-0.483815567668126,
-0.434914230461427,-0.399786211719122,-0.395498602433246,-0.392959614744107,
-0.391019331782558,-0.388945197683011,-0.385692633640207,-0.37534745817258,
-0.358709933410719,-0.325788728069424,-0.307655482357201,-0.290153304075602,
-0.287476857138846,-0.286117435821882,-0.285045331244668,-0.283797813777857,
-0.281565897735133,-0.270936652621915,-0.247581560903225,-0.191918008431791,
-0.184489505918061,-0.181533193263817,-0.17972387503256,-0.177894703239262,
-0.175384812180395,-0.170035012739241,-0.162922483422438,-0.145434472534502,
-0.0957467128170975,-0.0781669160271442,-0.0754878194857416,-0.0747633067458267),
 .UNSPECIFIED.);
#885=B_SPLINE_CURVE_WITH_KNOTS('',3,(#87042,#87043,#87044,#87045,#87046,
#87047,#87048,#87049,#87050,#87051,#87052,#87053,#87054,#87055,#87056,#87057,
#87058,#87059,#87060,#87061,#87062,#87063,#87064,#87065,#87066,#87067,#87068,
#87069,#87070,#87071,#87072,#87073,#87074,#87075,#87076,#87077,#87078,#87079,
#87080,#87081,#87082,#87083,#87084,#87085,#87086,#87087,#87088,#87089,#87090,
#87091,#87092,#87093,#87094,#87095,#87096,#87097,#87098,#87099,#87100,#87101,
#87102,#87103,#87104,#87105,#87106,#87107,#87108,#87109,#87110,#87111,#87112,
#87113,#87114,#87115,#87116,#87117,#87118,#87119,#87120,#87121,#87122,#87123,
#87124,#87125,#87126,#87127,#87128,#87129,#87130,#87131,#87132,#87133,#87134,
#87135,#87136,#87137,#87138,#87139,#87140,#87141,#87142,#87143,#87144,#87145,
#87146,#87147,#87148,#87149,#87150,#87151,#87152,#87153,#87154,#87155,#87156,
#87157,#87158,#87159,#87160,#87161,#87162,#87163,#87164,#87165,#87166,#87167,
#87168,#87169,#87170,#87171,#87172,#87173,#87174,#87175,#87176,#87177,#87178,
#87179,#87180,#87181,#87182,#87183,#87184,#87185,#87186,#87187,#87188,#87189,
#87190,#87191,#87192,#87193,#87194,#87195,#87196,#87197,#87198,#87199,#87200,
#87201,#87202,#87203,#87204,#87205,#87206,#87207,#87208,#87209,#87210,#87211,
#87212,#87213,#87214,#87215,#87216,#87217,#87218,#87219,#87220,#87221,#87222,
#87223,#87224,#87225,#87226,#87227,#87228,#87229,#87230,#87231,#87232,#87233,
#87234,#87235,#87236,#87237,#87238,#87239,#87240,#87241,#87242,#87243,#87244,
#87245,#87246,#87247,#87248,#87249,#87250,#87251,#87252,#87253,#87254,#87255,
#87256,#87257,#87258,#87259,#87260,#87261,#87262,#87263,#87264,#87265,#87266,
#87267,#87268,#87269,#87270,#87271,#87272,#87273,#87274,#87275,#87276,#87277,
#87278,#87279,#87280,#87281,#87282,#87283,#87284,#87285,#87286,#87287,#87288,
#87289,#87290,#87291,#87292,#87293,#87294,#87295,#87296,#87297,#87298,#87299,
#87300,#87301,#87302,#87303,#87304,#87305,#87306,#87307,#87308,#87309,#87310,
#87311),.UNSPECIFIED.,.F.,.F.,(4,2,2,2,2,2,2,2,2,2,2,2,2,2,2,2,2,2,2,2,
2,2,2,2,2,2,2,2,2,2,2,2,2,2,2,2,2,2,2,2,2,2,2,2,2,2,2,2,2,2,2,2,2,2,2,2,
2,2,2,2,2,2,2,2,2,2,2,2,2,2,2,2,2,2,2,2,2,2,2,2,2,2,2,2,2,2,2,2,2,2,2,2,
2,2,2,2,2,2,2,2,2,2,2,2,2,2,2,2,2,2,2,2,2,2,2,2,2,2,2,2,2,2,2,2,2,2,2,2,
2,2,2,2,2,2,4),(-2.59336156192323,-2.57478143052137,-2.55593934383233,-2.54664458212764,
-2.54450174744568,-2.54327364423961,-2.54219865697171,-2.54080983467589,
-2.53789503501006,-2.50819909521878,-2.45775098895474,-2.44826218015948,
-2.44365500757166,-2.43987599389533,-2.43770533927899,-2.43768964522469,
-2.43767339861842,-2.4376565793801,-2.43763916662259,-2.4376211387297,-2.43760247330996,
-2.43758314717443,-2.4375631362795,-2.43754241572724,-2.43752095971209,
-2.43749874147679,-2.43747573263685,-2.43745569688231,-2.43743234721676,
-2.43740514153362,-2.43737345187315,-2.43733655193289,-2.43729360345781,
-2.43723939236148,-2.43529871969985,-2.43275677192872,-2.42845870417978,
-2.39333805620597,-2.34438012315355,-2.33468140182116,-2.33251030840455,
-2.33127611547429,-2.33020231057727,-2.32882355086259,-2.3259595807232,
-2.29000856849919,-2.25724261206533,-2.23468164815311,-2.22902810391243,
-2.22645693900437,-2.22451860391383,-2.22269203547157,-2.22015033129157,
-2.21351002015316,-2.15770272017822,-2.13364361485811,-2.12282133203953,
-2.12057750414133,-2.11932733480963,-2.11825542928027,-2.11689943314798,
-2.11475392602736,-2.10371704588551,-2.05250246420806,-2.02379370546777,
-2.01736014566069,-2.01465154303585,-2.01268993094642,-2.01089740094624,
-2.00803261471736,-2.00114866010443,-1.94807395082249,-1.92216817173204,
-1.91086149371006,-1.90858910201151,-1.90733273324799,-1.90626143377121,
-1.90491375171595,-1.90229224110401,-1.8862505578491,-1.8809612549938,-1.86637614080143,
-1.83348514191239,-1.81691872735997,-1.80660660076346,-1.80335773302879,
-1.80128435485331,-1.79934365526262,-1.79680250289913,-1.7925076421135,
-1.75739675969618,-1.708494036339,-1.69872315354024,-1.69654695124879,-1.69531155671128,
-1.69423779681118,-1.69286052051344,-1.69000454240626,-1.66720803090501,
-1.61159834211153,-1.59558698556985,-1.59181759916656,-1.58962918187653,
-1.58771503082604,-1.58534582137417,-1.58171257528808,-1.56461629029267,
-1.55654719992905,-1.52173742237,-1.49768870195535,-1.48686947392944,-1.4846259238267,
-1.48337585942629,-1.48230401313248,-1.48094805250604,-1.47828783658503,
-1.46123461091314,-1.44262325791515,-1.40966792875342,-1.39302313838362,
-1.38267571410956,-1.37942287949061,-1.37734868383741,-1.37540842168779,
-1.37286957539999,-1.36858249232163,-1.3340022010121,-1.27803793126164,
-1.27376421689344,-1.27209268463666,-1.27108068241409,-1.26997837560242,
-1.26841349788512,-1.26450107762448,-1.2598478307819),.UNSPECIFIED.);
#886=B_SPLINE_CURVE_WITH_KNOTS('',3,(#87317,#87318,#87319,#87320,#87321,
#87322,#87323,#87324,#87325,#87326,#87327,#87328,#87329,#87330,#87331,#87332,
#87333,#87334),.UNSPECIFIED.,.F.,.F.,(4,2,2,2,2,2,2,2,4),(-0.0751187453612548,
-0.0651105012340861,-0.06037386076549,-0.0579480733786947,-0.0560290630418665,
-0.0538783933071959,-0.0516516907416782,-0.0483298715753922,-0.000628983619687466),
 .UNSPECIFIED.);
#887=B_SPLINE_CURVE_WITH_KNOTS('',3,(#87335,#87336,#87337,#87338,#87339,
#87340,#87341,#87342,#87343,#87344,#87345,#87346,#87347,#87348,#87349,#87350,
#87351,#87352,#87353,#87354,#87355,#87356,#87357,#87358,#87359,#87360,#87361,
#87362,#87363,#87364,#87365,#87366,#87367,#87368,#87369,#87370,#87371,#87372,
#87373,#87374,#87375,#87376,#87377,#87378,#87379,#87380,#87381,#87382,#87383,
#87384,#87385,#87386,#87387,#87388,#87389,#87390,#87391,#87392,#87393,#87394,
#87395,#87396,#87397,#87398,#87399,#87400,#87401,#87402,#87403,#87404,#87405,
#87406,#87407,#87408,#87409,#87410,#87411,#87412,#87413,#87414,#87415,#87416,
#87417,#87418,#87419,#87420,#87421,#87422,#87423,#87424,#87425,#87426,#87427,
#87428,#87429,#87430,#87431,#87432,#87433,#87434,#87435,#87436,#87437,#87438,
#87439,#87440,#87441,#87442,#87443,#87444,#87445,#87446,#87447,#87448,#87449,
#87450,#87451,#87452,#87453,#87454,#87455,#87456,#87457,#87458,#87459,#87460,
#87461,#87462,#87463,#87464,#87465,#87466,#87467,#87468,#87469,#87470,#87471,
#87472,#87473,#87474,#87475,#87476,#87477,#87478,#87479,#87480,#87481,#87482,
#87483,#87484,#87485,#87486,#87487,#87488,#87489,#87490,#87491,#87492,#87493,
#87494,#87495,#87496,#87497,#87498,#87499,#87500,#87501,#87502,#87503,#87504,
#87505,#87506,#87507,#87508,#87509,#87510,#87511,#87512,#87513,#87514,#87515,
#87516,#87517,#87518,#87519,#87520,#87521,#87522,#87523,#87524,#87525,#87526,
#87527,#87528,#87529,#87530,#87531,#87532,#87533,#87534,#87535,#87536,#87537,
#87538,#87539,#87540,#87541,#87542,#87543,#87544,#87545,#87546,#87547,#87548,
#87549,#87550,#87551,#87552,#87553,#87554,#87555,#87556),.UNSPECIFIED.,
 .F.,.F.,(4,2,2,2,2,2,2,2,2,2,2,2,2,2,2,2,2,2,2,2,2,2,2,2,2,2,2,2,2,2,2,
2,2,2,2,2,2,2,2,2,2,2,2,2,2,2,2,2,2,2,2,2,2,2,2,2,2,2,2,2,2,2,2,2,2,2,2,
2,2,2,2,2,2,2,2,2,2,2,2,2,2,2,2,2,2,2,2,2,2,2,2,2,2,2,2,2,2,2,2,2,2,2,2,
2,2,2,2,2,2,2,4),(-2.66770883390819,-2.62475437947397,-2.62182039698666,
-2.62013764316661,-2.61863271120716,-2.61754110563343,-2.61651378655355,
-2.61476419075559,-2.60998994102848,-2.57253353119947,-2.55111147084882,
-2.52277528452494,-2.5163024293871,-2.51417823115161,-2.51209832105435,
-2.51015950891412,-2.50763229531544,-2.50338650214394,-2.47116894427638,
-2.43568387162433,-2.41824496460406,-2.40942522411099,-2.4073250254246,
-2.40609673682713,-2.40502162768412,-2.40363270124937,-2.40071787126955,
-2.37055198924443,-2.31898104760483,-2.31037045964199,-2.30414811920189,
-2.30144314075866,-2.29948181255181,-2.29768792960418,-2.29481746895974,
-2.28790168012843,-2.23521529940548,-2.20902243734717,-2.19764164563069,
-2.1953645979624,-2.19410702490264,-2.1930355290242,-2.19168865638841,-2.18907182343594,
-2.17312088523044,-2.16870947085322,-2.1212960017337,-2.09763170555318,
-2.09182996308736,-2.08923137140871,-2.08728831601194,-2.08546889697837,
-2.08295556451277,-2.07649410279332,-2.01901926601932,-2.01352901529623,
-1.99464804991438,-1.98534047415626,-1.98319650409771,-1.98196804304497,
-1.9808929335475,-1.97950420539227,-1.97659049297645,-1.94574484197275,
-1.91160705879477,-1.89279440974746,-1.88149507036608,-1.87813705797889,
-1.87603926792662,-1.87410658231444,-1.87161933169763,-1.86751013870077,
-1.84101288018382,-1.7987996740724,-1.78190320528097,-1.77324605356108,
-1.77115096679496,-1.76993330747051,-1.76885618478708,-1.76747291670273,
-1.76518837826371,-1.75160543176326,-1.74979161422262,-1.70241888116661,
-1.67144365740888,-1.66699164886286,-1.66465602632956,-1.66274353610972,
-1.66052856524602,-1.65674101830539,-1.64214654861088,-1.62988100369963,
-1.58946989164561,-1.57061614481818,-1.56131733084317,-1.55917404804256,
-1.55794576633558,-1.55687067391552,-1.55548178319651,-1.5525670779959,
-1.52372979537384,-1.48561863062846,-1.46809306001602,-1.45735195754653,
-1.45405428450517,-1.45196987343531,-1.45003278989325,-1.44751625700801,
-1.44330699841092,-1.41283233438342,-1.4084593254711),.UNSPECIFIED.);
#888=B_SPLINE_CURVE_WITH_KNOTS('',3,(#87558,#87559,#87560,#87561,#87562,
#87563,#87564,#87565,#87566,#87567,#87568,#87569,#87570,#87571,#87572,#87573,
#87574,#87575,#87576,#87577,#87578,#87579,#87580,#87581,#87582,#87583,#87584,
#87585,#87586,#87587,#87588,#87589,#87590,#87591,#87592,#87593,#87594,#87595,
#87596,#87597,#87598,#87599,#87600,#87601,#87602,#87603,#87604,#87605,#87606,
#87607,#87608,#87609,#87610,#87611,#87612,#87613,#87614,#87615,#87616,#87617,
#87618,#87619,#87620,#87621,#87622,#87623,#87624,#87625,#87626,#87627,#87628,
#87629,#87630,#87631,#87632,#87633,#87634,#87635,#87636,#87637,#87638,#87639,
#87640,#87641,#87642,#87643,#87644,#87645,#87646,#87647,#87648,#87649,#87650,
#87651,#87652,#87653,#87654,#87655,#87656,#87657,#87658,#87659,#87660,#87661,
#87662,#87663,#87664,#87665,#87666,#87667,#87668,#87669,#87670,#87671,#87672,
#87673,#87674,#87675,#87676,#87677,#87678,#87679,#87680,#87681,#87682,#87683,
#87684,#87685,#87686,#87687,#87688,#87689,#87690,#87691,#87692,#87693,#87694,
#87695,#87696,#87697,#87698,#87699,#87700,#87701,#87702,#87703,#87704,#87705,
#87706,#87707,#87708,#87709,#87710,#87711,#87712,#87713,#87714,#87715,#87716,
#87717,#87718,#87719,#87720,#87721,#87722,#87723,#87724,#87725,#87726,#87727,
#87728,#87729,#87730,#87731,#87732,#87733,#87734,#87735,#87736,#87737,#87738,
#87739,#87740,#87741,#87742,#87743,#87744,#87745,#87746,#87747,#87748,#87749,
#87750,#87751,#87752,#87753,#87754,#87755,#87756,#87757,#87758,#87759,#87760,
#87761,#87762,#87763,#87764,#87765,#87766,#87767,#87768,#87769,#87770,#87771,
#87772,#87773,#87774,#87775,#87776,#87777,#87778,#87779,#87780,#87781,#87782,
#87783,#87784,#87785,#87786,#87787,#87788,#87789,#87790,#87791,#87792,#87793,
#87794,#87795,#87796,#87797,#87798,#87799,#87800,#87801,#87802,#87803,#87804,
#87805,#87806,#87807,#87808,#87809,#87810,#87811,#87812,#87813,#87814,#87815,
#87816,#87817,#87818,#87819,#87820,#87821,#87822,#87823,#87824,#87825,#87826,
#87827,#87828,#87829),.UNSPECIFIED.,.F.,.F.,(4,2,2,2,2,2,2,2,2,2,2,2,2,
2,2,2,2,2,2,2,2,2,2,2,2,2,2,2,2,2,2,2,2,2,2,2,2,2,2,2,2,2,2,2,2,2,2,2,2,
2,2,2,2,2,2,2,2,2,2,2,2,2,2,2,2,2,2,2,2,2,2,2,2,2,2,2,2,2,2,2,2,2,2,2,2,
2,2,2,2,2,2,2,2,2,2,2,2,2,2,2,2,2,2,2,2,2,2,2,2,2,2,2,2,2,2,2,2,2,2,2,2,
2,2,2,2,2,2,2,2,2,2,2,2,2,2,4),(-1.2598478307819,-1.24528929234835,-1.1889169518329,
-1.17207227593167,-1.16845566072013,-1.16609162636776,-1.16417788367051,
-1.16198579247119,-1.15819960366846,-1.14195347226029,-1.08448120487193,
-1.07950865620043,-1.0635235292766,-1.06090524041075,-1.05955822062563,
-1.05848692416541,-1.05722995783808,-1.05495494653949,-1.04360421005489,
-1.01752345922582,-0.964653835092965,-0.957751193963408,-0.954883266774759,
-0.953090119321,-0.951128920320106,-0.948422876009794,-0.942004785276161,
-0.91343052938435,-0.862235796005543,-0.85107622247357,-0.848923187726734,
-0.847564892259753,-0.846492810145333,-0.845244325579734,-0.843008214191392,
-0.832312720154088,-0.808717499380194,-0.752157189499822,-0.74559191523724,
-0.743062108439144,-0.741238682966653,-0.73929868715275,-0.736716775439302,
-0.731004511911674,-0.708010054349212,-0.674995329328759,-0.65397405074336,
-0.639432548045239,-0.637102678852817,-0.635706346157752,-0.634627890714361,
-0.633418611436055,-0.631359981455373,-0.623149413636835,-0.607538527463072,
-0.565819259417715,-0.537126733153774,-0.532961633694862,-0.530458475445625,
-0.52852400770821,-0.526434805620254,-0.523113253335846,-0.512147136109772,
-0.494107901067988,-0.443946508571429,-0.427608372243173,-0.424975729079608,
-0.42362570905684,-0.422554323276223,-0.42129990873719,-0.419036243486443,
-0.407878555369356,-0.382547883822278,-0.328603155968634,-0.32178776827569,
-0.318934408159038,-0.317144042427059,-0.315180779553109,-0.312462489029747,
-0.30597053637577,-0.29698364226265,-0.245936659350276,-0.215997823684719,
-0.213149026927364,-0.211767348847781,-0.210714957827224,-0.210704912418351,
-0.210695176616752,-0.210685727169198,-0.210676543231602,-0.210667605835312,
-0.210658897893402,-0.210650403950862,-0.210642109808122,-0.210634002554713,
-0.210626070366007,-0.210618302312035,-0.210610688405847,-0.210603219397911,
-0.210595886676978,-0.21058868220452,-0.210581598612733,-0.210574629069274,
-0.210567767032783,-0.210561006531983,-0.210554341949679,-0.2105477679807,
-0.210541279592807,-0.210534872074776,-0.21052854103106,-0.21052228227184,
-0.210516091863237,-0.210509966007037,-0.210503901164927,-0.210497893989959,
-0.210491941191575,-0.210486039768665,-0.210480186773141,-0.210474379385115,
-0.209210206527847,-0.206817809032165,-0.193151295846991,-0.156400889779779,
-0.113382385035125,-0.109096409479968,-0.106558041419045,-0.104618031374231,
-0.102543994241103,-0.0992911748388577,-0.0889417362901918,-0.0722940605167449,
-0.0417947654359074,-0.00539400818564538,-0.00193479222001944,-0.000864069735648079,
-0.000629066024222938),.UNSPECIFIED.);
#889=B_SPLINE_CURVE_WITH_KNOTS('',3,(#87830,#87831,#87832,#87833,#87834,
#87835,#87836,#87837,#87838,#87839,#87840,#87841,#87842,#87843,#87844,#87845),
 .UNSPECIFIED.,.F.,.F.,(4,3,3,3,3,4),(-28.973780262141,-28.9662570488944,
-28.8628842312553,-28.7596459044043,-28.6565264336762,-28.6232428001367),
 .UNSPECIFIED.);
#890=B_SPLINE_CURVE_WITH_KNOTS('',3,(#87850,#87851,#87852,#87853,#87854,
#87855,#87856,#87857,#87858,#87859,#87860,#87861,#87862,#87863,#87864,#87865,
#87866,#87867,#87868,#87869,#87870,#87871,#87872,#87873,#87874,#87875,#87876,
#87877,#87878,#87879,#87880,#87881,#87882,#87883,#87884,#87885,#87886,#87887,
#87888,#87889,#87890,#87891,#87892,#87893,#87894,#87895,#87896,#87897,#87898,
#87899,#87900,#87901,#87902,#87903,#87904,#87905,#87906,#87907,#87908,#87909,
#87910,#87911,#87912,#87913,#87914,#87915,#87916,#87917,#87918,#87919,#87920,
#87921,#87922,#87923,#87924,#87925,#87926,#87927,#87928,#87929,#87930,#87931,
#87932,#87933,#87934,#87935,#87936,#87937,#87938,#87939,#87940,#87941,#87942,
#87943,#87944,#87945,#87946,#87947,#87948,#87949,#87950,#87951,#87952,#87953,
#87954,#87955,#87956,#87957,#87958,#87959,#87960,#87961,#87962,#87963,#87964,
#87965,#87966,#87967,#87968,#87969,#87970,#87971,#87972,#87973,#87974,#87975,
#87976,#87977,#87978,#87979,#87980,#87981,#87982,#87983,#87984,#87985,#87986,
#87987,#87988,#87989,#87990,#87991,#87992,#87993,#87994,#87995,#87996,#87997,
#87998,#87999,#88000,#88001,#88002,#88003,#88004,#88005,#88006,#88007,#88008,
#88009,#88010,#88011,#88012,#88013,#88014,#88015,#88016,#88017,#88018,#88019,
#88020,#88021,#88022,#88023,#88024,#88025,#88026,#88027,#88028,#88029,#88030,
#88031,#88032,#88033,#88034,#88035,#88036,#88037,#88038,#88039,#88040,#88041,
#88042,#88043,#88044,#88045,#88046,#88047,#88048,#88049,#88050,#88051,#88052,
#88053,#88054,#88055,#88056,#88057,#88058,#88059,#88060,#88061,#88062,#88063,
#88064,#88065,#88066,#88067,#88068,#88069,#88070,#88071,#88072,#88073,#88074,
#88075,#88076,#88077,#88078,#88079),.UNSPECIFIED.,.F.,.F.,(4,2,2,2,2,2,
2,2,2,2,2,2,2,2,2,2,2,2,2,2,2,2,2,2,2,2,2,2,2,2,2,2,2,2,2,2,2,2,2,2,2,2,
2,2,2,2,2,2,2,2,2,2,2,2,2,2,2,2,2,2,2,2,2,2,2,2,2,2,2,2,2,2,2,2,2,2,2,2,
2,2,2,2,2,2,2,2,2,2,2,2,2,2,2,2,2,2,2,2,2,2,2,2,2,2,2,2,2,2,2,2,2,2,2,2,
4),(-1.40850153180492,-1.36250266792624,-1.34494718878491,-1.33419300667973,
-1.33089396069365,-1.32880929375025,-1.32687239494307,-1.32431321406307,
-1.31872670134852,-1.31130334259201,-1.29270174146163,-1.24997366761145,
-1.2273458145331,-1.22449368388517,-1.2231170476229,-1.22204321147614,-1.22080708773443,
-1.21862805117604,-1.20881907582038,-1.15991453630915,-1.12479584722585,
-1.12050022469114,-1.11795871973547,-1.11601779643587,-1.11394422253493,
-1.11069513726152,-1.10038298714613,-1.08381947663768,-1.05095674662274,
-1.03712853846431,-1.03047927309802,-1.01500557839671,-1.01240852061588,
-1.01106603294309,-1.00999495536059,-1.00873430560225,-1.00644253944657,
-0.994796209914545,-0.967531040131002,-0.947346484138139,-0.912838732964867,
-0.908552107360215,-0.906013234804672,-0.904072770255018,-0.90199818027652,
-0.898744353772751,-0.888390524142,-0.871734651222027,-0.838795741074562,
-0.82007236579395,-0.803159000758074,-0.800503827905399,-0.799148848740516,
-0.798076953647933,-0.796825889660074,-0.79457817768722,-0.783693760074211,
-0.759401953478156,-0.703899695701145,-0.697224656244714,-0.694677436365725,
-0.692849337799291,-0.690911613820067,-0.688345046551784,-0.682716977631982,
-0.67522336157879,-0.65636360023919,-0.626448513375451,-0.604721939855228,
-0.590952696337158,-0.588659664226564,-0.587274112310235,-0.586196990964432,
-0.584981347491901,-0.582894265567584,-0.57433331247896,-0.557714673050792,
-0.51552930042313,-0.48862337974378,-0.484504558176909,-0.482014905507422,
-0.480082380799827,-0.477986794396815,-0.474636721032121,-0.463405649177908,
-0.444752960510814,-0.416482353160889,-0.379486197159405,-0.376648554453402,
-0.375274992402946,-0.374201702432199,-0.372964110749879,-0.370777445489433,
-0.361223097587746,-0.312152855856071,-0.276986607863795,-0.272691418201515,
-0.270150396569206,-0.268209973218679,-0.26613706028445,-0.262889275515635,
-0.25277870278595,-0.236574232997193,-0.198328815996906,-0.167652335617237,
-0.164739946834172,-0.163351838439206,-0.16227719980241,-0.161049276032689,
-0.159757267485298,-0.155110071347819,-0.128864883232683,-0.106990879308478,
-0.105559660604484,-0.0751187453612548),.UNSPECIFIED.);
#891=B_SPLINE_CURVE_WITH_KNOTS('',3,(#88081,#88082,#88083,#88084,#88085,
#88086,#88087,#88088,#88089,#88090,#88091,#88092,#88093,#88094,#88095,#88096,
#88097,#88098,#88099,#88100,#88101,#88102,#88103,#88104,#88105,#88106,#88107,
#88108,#88109,#88110,#88111,#88112,#88113,#88114,#88115,#88116,#88117,#88118,
#88119,#88120,#88121,#88122,#88123,#88124,#88125,#88126,#88127,#88128,#88129,
#88130,#88131,#88132,#88133,#88134,#88135,#88136,#88137,#88138,#88139,#88140,
#88141,#88142,#88143,#88144,#88145,#88146,#88147,#88148,#88149,#88150,#88151,
#88152,#88153,#88154,#88155,#88156,#88157,#88158,#88159,#88160,#88161,#88162,
#88163,#88164,#88165,#88166,#88167,#88168,#88169,#88170,#88171,#88172,#88173,
#88174,#88175,#88176,#88177,#88178,#88179,#88180,#88181,#88182,#88183,#88184,
#88185,#88186,#88187,#88188,#88189,#88190,#88191,#88192,#88193,#88194,#88195,
#88196,#88197,#88198,#88199,#88200,#88201,#88202,#88203,#88204,#88205,#88206,
#88207,#88208,#88209,#88210,#88211,#88212,#88213,#88214,#88215,#88216,#88217,
#88218,#88219,#88220,#88221,#88222,#88223,#88224,#88225,#88226,#88227,#88228,
#88229,#88230,#88231,#88232,#88233,#88234,#88235,#88236,#88237,#88238,#88239,
#88240,#88241,#88242,#88243,#88244,#88245,#88246,#88247,#88248,#88249,#88250,
#88251,#88252,#88253,#88254,#88255,#88256,#88257,#88258,#88259,#88260,#88261),
 .UNSPECIFIED.,.F.,.F.,(4,3,3,3,3,3,3,3,3,3,3,3,3,3,3,3,3,3,3,3,3,3,3,3,
3,3,3,3,3,3,3,3,3,3,3,3,3,3,3,3,3,3,3,3,3,3,3,3,3,3,3,3,3,3,3,3,3,3,3,3,
4),(-28.6232428001367,-28.5202020676114,-28.4171817229006,-28.3141477785777,
-28.2110001876892,-28.1077864190661,-28.0043998217136,-27.9674205989325,
-27.864025861899,-27.7607845797985,-27.657664614421,-27.554610046227,-27.4515868378843,
-27.348560995227,-27.245428228464,-27.1422391370694,-27.0388671437028,-26.9685841489706,
-26.8651894118465,-26.7619481296552,-26.6588281641867,-26.5557735959016,
-26.452750387468,-26.3497245447198,-26.2465917778671,-26.1434026863831,
-26.0400306929288,-25.9697476990087,-25.8663529620659,-25.7631116800558,
-25.6599917147673,-25.5569371466616,-25.4539139384064,-25.3508880958353,
-25.2477553291566,-25.1445662378452,-25.0411942445592,-24.9709112490469,
-24.8675165120623,-24.764275230012,-24.6611552646861,-24.5581006965446,
-24.4550774882552,-24.3520516456518,-24.2489188789436,-24.1457297876041,
-24.0423577942929,-23.972074799085,-23.8686800615146,-23.7654387788755,
-23.6623188129591,-23.5592642442264,-23.4562410353459,-23.3532151921524,
-23.2500824248597,-23.146893332938,-23.0435213390546,-22.9732383491231,
-22.8444301460866,-22.7177283293138,-22.6905949549614),.UNSPECIFIED.);
#892=B_SPLINE_CURVE_WITH_KNOTS('',3,(#88262,#88263,#88264,#88265),
 .UNSPECIFIED.,.F.,.F.,(4,4),(-22.6905949549614,-22.3411472771506),
 .UNSPECIFIED.);
#893=B_SPLINE_CURVE_WITH_KNOTS('',3,(#88271,#88272,#88273,#88274,#88275,
#88276,#88277,#88278,#88279,#88280,#88281,#88282,#88283,#88284,#88285,#88286,
#88287,#88288),.UNSPECIFIED.,.F.,.F.,(4,2,2,2,2,2,2,2,4),(-0.0747374473528612,
-0.04412382595158,-0.0412117156485017,-0.0398236209285753,-0.0387489379637731,
-0.0375209019896154,-0.036228756208033,-0.0342507643538522,-0.000628700947229318),
 .UNSPECIFIED.);
#894=B_SPLINE_CURVE_WITH_KNOTS('',3,(#88289,#88290,#88291,#88292,#88293,
#88294,#88295,#88296,#88297,#88298,#88299,#88300,#88301,#88302,#88303,#88304,
#88305,#88306,#88307,#88308,#88309,#88310,#88311,#88312,#88313,#88314,#88315,
#88316,#88317,#88318,#88319,#88320,#88321,#88322,#88323,#88324,#88325,#88326,
#88327,#88328,#88329,#88330,#88331,#88332,#88333,#88334,#88335,#88336,#88337,
#88338,#88339,#88340,#88341,#88342,#88343,#88344,#88345,#88346,#88347,#88348,
#88349,#88350,#88351,#88352,#88353,#88354,#88355,#88356,#88357,#88358,#88359,
#88360,#88361,#88362,#88363,#88364,#88365,#88366,#88367,#88368,#88369,#88370,
#88371,#88372,#88373,#88374,#88375,#88376,#88377,#88378,#88379,#88380,#88381,
#88382,#88383,#88384,#88385,#88386,#88387,#88388,#88389,#88390,#88391,#88392,
#88393,#88394,#88395,#88396,#88397,#88398,#88399,#88400,#88401,#88402,#88403,
#88404,#88405,#88406,#88407,#88408,#88409,#88410,#88411,#88412,#88413,#88414,
#88415,#88416,#88417,#88418,#88419,#88420,#88421,#88422,#88423,#88424,#88425,
#88426,#88427,#88428,#88429,#88430,#88431,#88432,#88433,#88434,#88435,#88436,
#88437,#88438,#88439,#88440,#88441,#88442,#88443,#88444,#88445,#88446,#88447,
#88448,#88449,#88450,#88451,#88452,#88453,#88454,#88455,#88456,#88457,#88458,
#88459,#88460,#88461,#88462,#88463,#88464,#88465,#88466,#88467,#88468,#88469,
#88470,#88471,#88472,#88473,#88474,#88475,#88476,#88477,#88478,#88479,#88480,
#88481,#88482,#88483,#88484,#88485,#88486,#88487,#88488,#88489,#88490,#88491,
#88492,#88493,#88494,#88495,#88496,#88497,#88498,#88499,#88500,#88501,#88502,
#88503,#88504,#88505,#88506,#88507,#88508),.UNSPECIFIED.,.F.,.F.,(4,2,2,
2,2,2,2,2,2,2,2,2,2,2,2,2,2,2,2,2,2,2,2,2,2,2,2,2,2,2,2,2,2,2,2,2,2,2,2,
2,2,2,2,2,2,2,2,2,2,2,2,2,2,2,2,2,2,2,2,2,2,2,2,2,2,2,2,2,2,2,2,2,2,2,2,
2,2,2,2,2,2,2,2,2,2,2,2,2,2,2,2,2,2,2,2,2,2,2,2,2,2,2,2,2,2,2,2,2,2,4),
(-2.66802904969001,-2.63755774389658,-2.6110418457987,-2.60487466067178,
-2.60221136333042,-2.60025753768377,-2.59845461781743,-2.59553444665161,
-2.58831963533694,-2.54291704431415,-2.52278593755294,-2.50657158531799,
-2.49817521853025,-2.49612782426245,-2.49489968701426,-2.49382468719195,
-2.49243587130156,-2.48952116456729,-2.45949023876327,-2.40819232067015,
-2.39936297756314,-2.39296024987529,-2.39025661551927,-2.38829568401878,
-2.38650176556769,-2.38363037935178,-2.37670786679604,-2.324126944789,-2.29786687814242,
-2.28646960463217,-2.28419178777279,-2.28293412750553,-2.28186276177362,
-2.28051631274538,-2.27790106567353,-2.26197752629999,-2.25748987063338,
-2.21495986223702,-2.18434884153593,-2.17990718751521,-2.17757390691457,
-2.17566176417161,-2.17344542745107,-2.16965122176219,-2.15497798465485,
-2.14272683561657,-2.10721237745275,-2.08476869321325,-2.07439290602801,
-2.07217670138004,-2.07093249920516,-2.06985983366734,-2.0684952881174,
-2.06579533980039,-2.04761467920952,-2.02952801031757,-1.99679796239865,
-1.97429793992573,-1.96865218839525,-1.96608218613366,-1.96414375748969,
-1.96231638762754,-1.9597724228585,-1.9531193589139,-1.8974130695201,-1.87327725586826,
-1.86243353454152,-1.86018812810855,-1.85893748043094,-1.85786541198845,
-1.85650952682316,-1.85436478916682,-1.84334447379542,-1.79204460878004,
-1.76337818485223,-1.75694913947586,-1.75424101398548,-1.75227923067451,
-1.75048618869259,-1.74761981083507,-1.74072802435933,-1.68773031081081,
-1.66175996773514,-1.65043601167667,-1.64816234295048,-1.64690556307631,
-1.645834092069,-1.64448642212537,-1.64186560534487,-1.62583988317903,-1.62044303705025,
-1.60593861968782,-1.57304280848175,-1.5502861793192,-1.54460557757692,
-1.54202907056096,-1.5400895318011,-1.53826389985079,-1.53572681601022,
-1.52911815609688,-1.47296827102802,-1.44911913430193,-1.43835263235197,
-1.43611180790494,-1.43486210661223,-1.43378985815367,-1.43243247262926,
-1.42976671205318,-1.41257999831609,-1.40850153180492),.UNSPECIFIED.);
#895=B_SPLINE_CURVE_WITH_KNOTS('',3,(#88510,#88511,#88512,#88513,#88514,
#88515,#88516,#88517,#88518,#88519),.UNSPECIFIED.,.F.,.F.,(4,1,1,1,1,1,
1,4),(-22.3411472771506,-21.9744018991612,-20.9755654491994,-19.9767289992375,
-18.9778925492756,-17.9790560993137,-16.9802196493519,-16.4074096477818),
 .UNSPECIFIED.);
#896=B_SPLINE_CURVE_WITH_KNOTS('',3,(#88520,#88521,#88522,#88523,#88524,
#88525),.UNSPECIFIED.,.F.,.F.,(4,2,4),(-2.66742168930548,-2.60891632352633,
-2.59315595267277),.UNSPECIFIED.);
#897=B_SPLINE_CURVE_WITH_KNOTS('',3,(#88530,#88531,#88532,#88533,#88534,
#88535,#88536,#88537,#88538,#88539,#88540,#88541,#88542,#88543,#88544,#88545,
#88546,#88547,#88548,#88549,#88550,#88551,#88552,#88553,#88554,#88555,#88556,
#88557,#88558,#88559,#88560,#88561,#88562,#88563,#88564,#88565,#88566,#88567,
#88568,#88569,#88570,#88571,#88572,#88573,#88574,#88575,#88576,#88577,#88578,
#88579,#88580,#88581,#88582,#88583,#88584,#88585,#88586,#88587,#88588,#88589,
#88590,#88591,#88592,#88593,#88594,#88595,#88596,#88597,#88598,#88599,#88600,
#88601,#88602,#88603,#88604,#88605,#88606,#88607,#88608,#88609,#88610,#88611,
#88612,#88613,#88614,#88615,#88616,#88617,#88618,#88619,#88620,#88621,#88622,
#88623,#88624,#88625,#88626,#88627,#88628,#88629,#88630,#88631,#88632,#88633,
#88634,#88635,#88636,#88637,#88638,#88639,#88640,#88641,#88642,#88643,#88644,
#88645,#88646,#88647,#88648,#88649,#88650,#88651,#88652,#88653,#88654,#88655,
#88656,#88657,#88658,#88659,#88660,#88661,#88662,#88663,#88664,#88665,#88666,
#88667,#88668,#88669,#88670,#88671,#88672,#88673,#88674,#88675,#88676,#88677,
#88678,#88679,#88680,#88681,#88682,#88683,#88684,#88685,#88686,#88687,#88688,
#88689,#88690,#88691,#88692,#88693,#88694,#88695,#88696,#88697,#88698,#88699,
#88700,#88701,#88702,#88703,#88704,#88705,#88706,#88707,#88708,#88709,#88710,
#88711,#88712,#88713,#88714,#88715,#88716,#88717,#88718,#88719,#88720,#88721,
#88722,#88723,#88724,#88725,#88726,#88727,#88728,#88729,#88730,#88731,#88732,
#88733,#88734,#88735,#88736,#88737,#88738,#88739,#88740,#88741,#88742,#88743,
#88744,#88745,#88746,#88747,#88748,#88749,#88750,#88751,#88752,#88753,#88754,
#88755,#88756,#88757),.UNSPECIFIED.,.F.,.F.,(4,2,2,2,2,2,2,2,2,2,2,2,2,
2,2,2,2,2,2,2,2,2,2,2,2,2,2,2,2,2,2,2,2,2,2,2,2,2,2,2,2,2,2,2,2,2,2,2,2,
2,2,2,2,2,2,2,2,2,2,2,2,2,2,2,2,2,2,2,2,2,2,2,2,2,2,2,2,2,2,2,2,2,2,2,2,
2,2,2,2,2,2,2,2,2,2,2,2,2,2,2,2,2,2,2,2,2,2,2,2,2,2,2,2,4),(-1.40833650609706,
-1.3649437306449,-1.33389381709473,-1.31584387047142,-1.31314824084025,
-1.31178459144683,-1.31071196445864,-1.30946704779559,-1.30724773180197,
-1.29682452600705,-1.27421113791659,-1.21608710496737,-1.20970344861157,
-1.20720318981174,-1.20538733098271,-1.20344254810514,-1.20083203889336,
-1.19496299129987,-1.1707865138568,-1.12030328273454,-1.11987263331321,
-1.10368575152951,-1.10105877473431,-1.09970982450841,-1.09863833001689,
-1.09738268167455,-1.09511396777183,-1.08387445595086,-1.05823025922132,
-1.00472618569253,-0.997872335794782,-0.995012325098936,-0.993220533540396,
-0.991257922917696,-0.988544613707199,-0.982084031750929,-0.928143104171845,
-0.891939834625717,-0.889085064613198,-0.887708000231669,-0.886634227682866,
-0.885398626158178,-0.883221586824627,-0.873439475014806,-0.824518597785424,
-0.789396346049497,-0.785101093367893,-0.782559837634135,-0.780619122208955,
-0.778545787427025,-0.775297112459875,-0.764986566013361,-0.748425920597504,
-0.715567628486558,-0.701829267242749,-0.694974244682334,-0.694646738812136,
-0.688836527048918,-0.679050447296629,-0.676987308449316,-0.675656580996106,
-0.674586232869739,-0.673316269086304,-0.670980995979987,-0.658511789946157,
-0.601784247668701,-0.592637781831421,-0.576122516071506,-0.572529065390159,
-0.570172304108043,-0.568259201161152,-0.566062052669969,-0.562252383520181,
-0.545669852662471,-0.485258319331414,-0.46770889562479,-0.46503072363384,
-0.463670913620932,-0.462598753705616,-0.461351460183848,-0.459120655746634,
-0.448509962292842,-0.425222459498542,-0.368183702264911,-0.3616740559574,
-0.359153296358345,-0.357332297268636,-0.355391083321029,-0.352801024332959,
-0.347043664672101,-0.298622221255579,-0.296632139941095,-0.277730750328994,
-0.271008271974131,-0.255576068838208,-0.253209102980117,-0.251801933881499,
-0.250722003063835,-0.24951870369754,-0.247527743032982,-0.240021742540941,
-0.226283927436843,-0.195002955852307,-0.180519452277464,-0.153157428159492,
-0.149027139595264,-0.146534157834852,-0.144601186953499,-0.142507252777016,
-0.139164453911593,-0.128001196418437,-0.0983529125791534,-0.0750367835752176,
-0.0747374473528612),.UNSPECIFIED.);
#898=B_SPLINE_CURVE_WITH_KNOTS('',3,(#88758,#88759,#88760,#88761,#88762,
#88763,#88764,#88765,#88766,#88767,#88768,#88769,#88770,#88771,#88772,#88773,
#88774,#88775,#88776,#88777,#88778,#88779,#88780,#88781,#88782,#88783,#88784,
#88785,#88786,#88787,#88788,#88789,#88790,#88791,#88792,#88793,#88794,#88795,
#88796,#88797,#88798,#88799,#88800,#88801,#88802,#88803,#88804,#88805,#88806,
#88807,#88808,#88809,#88810,#88811,#88812,#88813,#88814,#88815,#88816,#88817,
#88818,#88819,#88820,#88821,#88822,#88823,#88824,#88825,#88826,#88827,#88828,
#88829,#88830,#88831,#88832,#88833,#88834,#88835,#88836,#88837,#88838,#88839,
#88840,#88841,#88842,#88843,#88844,#88845,#88846,#88847,#88848,#88849,#88850,
#88851,#88852,#88853,#88854,#88855,#88856,#88857,#88858,#88859,#88860,#88861,
#88862,#88863,#88864,#88865,#88866,#88867,#88868,#88869,#88870,#88871,#88872,
#88873,#88874,#88875,#88876,#88877,#88878,#88879,#88880,#88881,#88882,#88883,
#88884,#88885,#88886,#88887,#88888,#88889,#88890,#88891,#88892,#88893,#88894,
#88895,#88896,#88897,#88898,#88899,#88900,#88901,#88902,#88903,#88904,#88905,
#88906,#88907,#88908,#88909,#88910,#88911,#88912,#88913,#88914,#88915,#88916,
#88917,#88918,#88919,#88920,#88921,#88922,#88923,#88924,#88925,#88926,#88927,
#88928,#88929,#88930,#88931,#88932,#88933,#88934,#88935,#88936,#88937,#88938,
#88939,#88940,#88941,#88942,#88943,#88944,#88945,#88946,#88947,#88948,#88949,
#88950,#88951,#88952,#88953,#88954,#88955,#88956,#88957,#88958,#88959,#88960,
#88961,#88962,#88963,#88964,#88965,#88966,#88967,#88968,#88969,#88970,#88971,
#88972,#88973,#88974,#88975,#88976,#88977,#88978,#88979,#88980,#88981,#88982,
#88983,#88984,#88985,#88986,#88987,#88988,#88989,#88990,#88991),
 .UNSPECIFIED.,.F.,.F.,(4,2,2,2,2,2,2,2,2,2,2,2,2,2,2,2,2,2,2,2,2,2,2,2,
2,2,2,2,2,2,2,2,2,2,2,2,2,2,2,2,2,2,2,2,2,2,2,2,2,2,2,2,2,2,2,2,2,2,2,2,
2,2,2,2,2,2,2,2,2,2,2,2,2,2,2,2,2,2,2,2,2,2,2,2,2,2,2,2,2,2,2,2,2,2,2,2,
2,2,2,2,2,2,2,2,2,2,2,2,2,2,2,2,2,2,2,2,4),(-2.59315595267277,-2.59007765348889,
-2.58078448014978,-2.57864198523523,-2.57741407255166,-2.5763392499272,
-2.57495063749772,-2.57203626725213,-2.54226196803104,-2.49162801649512,
-2.48229546831666,-2.47774314132557,-2.47500475818302,-2.47252037497173,
-2.47064428591098,-2.46881788930564,-2.46627675620113,-2.45963991309685,
-2.40381682376284,-2.37976748382818,-2.36894790729867,-2.36670426759488,
-2.36545415076778,-2.36438225062132,-2.36302621301197,-2.36088056030463,
-2.34984120667498,-2.29863208912856,-2.26992327818169,-2.26348974737613,
-2.26078116271369,-2.25881956543299,-2.25702705011501,-2.25416228960172,
-2.24727840622048,-2.19420723025399,-2.1682997778496,-2.1569927404807,-2.15472034886713,
-2.15346398977869,-2.1523927173179,-2.15104508838411,-2.14842370523333,
-2.13238313327305,-2.12707697857598,-2.11250769039387,-2.07961732011986,
-2.06305117077562,-2.05273924478465,-2.04949046821774,-2.04741715562264,
-2.04547652282287,-2.04293546598963,-2.03864078566131,-2.00353527573851,
-1.95465270383452,-1.94486021660141,-1.9426825914827,-1.94144691070569,
-1.94037323520611,-1.93899650495304,-1.93614316750176,-1.91345110774454,
-1.87272400097021,-1.84568071029017,-1.83944854449809,-1.83677417344399,
-1.83481857270971,-1.83301845523671,-1.83011270095119,-1.82298260427717,
-1.77422260113915,-1.73505265691647,-1.73147802556188,-1.72996901940272,
-1.72887685602193,-1.72785086826456,-1.72610764576359,-1.7213745084549,
-1.6818016663528,-1.63388992437694,-1.62749311299658,-1.62479053606767,
-1.62282984421461,-1.62103578076845,-1.61816336590095,-1.61123424153424,
-1.55875510904605,-1.53242866434402,-1.52101503125635,-1.51873640051769,
-1.51747861786064,-1.51640744490045,-1.51506158223072,-1.51244823431088,
-1.49656815555236,-1.49069806144923,-1.4466670116864,-1.42810815085144,
-1.41691845241822,-1.41357285948488,-1.41147833394793,-1.40954560690936,
-1.40705404709314,-1.40292854555846,-1.37574265801168,-1.33373204453707,
-1.3276351152182,-1.30978754662863,-1.30709916239073,-1.30573723397509,
-1.30466495293353,-1.30341928395598,-1.30119586143113,-1.29070305718652,
-1.26784057085319,-1.25960927882884),.UNSPECIFIED.);
#899=B_SPLINE_CURVE_WITH_KNOTS('',3,(#88997,#88998,#88999,#89000,#89001,
#89002,#89003,#89004,#89005,#89006,#89007,#89008,#89009,#89010,#89011,#89012,
#89013,#89014,#89015,#89016,#89017,#89018,#89019,#89020,#89021,#89022,#89023,
#89024,#89025,#89026,#89027,#89028,#89029,#89030,#89031,#89032,#89033,#89034,
#89035,#89036,#89037,#89038,#89039,#89040,#89041,#89042,#89043,#89044,#89045,
#89046,#89047,#89048,#89049,#89050,#89051,#89052,#89053,#89054,#89055,#89056,
#89057,#89058,#89059,#89060,#89061,#89062,#89063,#89064,#89065,#89066,#89067,
#89068,#89069,#89070,#89071,#89072,#89073,#89074,#89075,#89076,#89077,#89078,
#89079,#89080,#89081,#89082,#89083,#89084,#89085,#89086,#89087,#89088,#89089,
#89090,#89091,#89092,#89093,#89094,#89095,#89096,#89097,#89098,#89099,#89100,
#89101,#89102),.UNSPECIFIED.,.F.,.F.,(4,3,3,3,3,3,3,3,3,3,3,3,3,3,3,3,3,
3,3,3,3,3,3,3,3,3,3,3,3,3,3,3,3,3,3,4),(-3.4905420525369,-3.38888724890093,
-3.28714616891576,-3.1853635306981,-3.08340260642831,-2.99650934988562,
-2.89298804639364,-2.7896177431212,-2.6863657748023,-2.58317744783227,-2.4800189405397,
-2.37685647276338,-2.2735860348565,-2.17025847843688,-2.06674831927576,
-1.99767289992375,-1.89536969270601,-1.79322053934975,-1.69118879043613,
-1.58921974834484,-1.48727804733066,-1.38532836211997,-1.28325632553546,
-1.18112129116516,-1.0787805560955,-0.998836449961877,-0.892562651586185,
-0.780992320137912,-0.67507184468024,-0.56925096547428,-0.463501942676278,
-0.357797126152519,-0.25207917949123,-0.14635615172218,-0.0405601678050039,
0.),.UNSPECIFIED.);
#900=B_SPLINE_CURVE_WITH_KNOTS('',3,(#89105,#89106,#89107,#89108,#89109,
#89110,#89111,#89112,#89113,#89114,#89115,#89116,#89117,#89118,#89119,#89120,
#89121,#89122,#89123,#89124,#89125,#89126,#89127,#89128,#89129,#89130,#89131,
#89132,#89133,#89134,#89135,#89136,#89137,#89138,#89139,#89140,#89141,#89142,
#89143,#89144,#89145,#89146,#89147,#89148,#89149,#89150,#89151,#89152,#89153,
#89154,#89155,#89156,#89157,#89158,#89159,#89160,#89161,#89162,#89163,#89164,
#89165,#89166,#89167,#89168,#89169,#89170,#89171,#89172,#89173,#89174,#89175,
#89176,#89177,#89178,#89179,#89180,#89181,#89182,#89183,#89184,#89185,#89186,
#89187,#89188,#89189,#89190,#89191,#89192,#89193,#89194,#89195,#89196,#89197,
#89198,#89199,#89200,#89201,#89202,#89203,#89204,#89205,#89206,#89207,#89208,
#89209,#89210,#89211,#89212,#89213,#89214,#89215,#89216,#89217,#89218,#89219,
#89220,#89221,#89222,#89223,#89224,#89225,#89226,#89227,#89228,#89229,#89230,
#89231,#89232,#89233,#89234,#89235,#89236,#89237,#89238,#89239,#89240,#89241,
#89242,#89243,#89244,#89245,#89246,#89247,#89248,#89249,#89250,#89251,#89252,
#89253,#89254,#89255,#89256,#89257,#89258,#89259,#89260,#89261,#89262,#89263,
#89264),.UNSPECIFIED.,.F.,.F.,(4,3,3,3,3,3,3,3,3,3,3,3,3,3,3,3,3,3,3,3,
3,3,3,3,3,3,3,3,3,3,3,3,3,3,3,3,3,3,3,3,3,3,3,3,3,3,3,3,3,3,3,3,3,4),(2.00878451784277,
2.11210385922517,2.21526978906692,2.31831430239263,2.42129361283959,2.52424186610781,
2.6271931648727,2.7302492654409,2.83336236205173,2.93665172410155,2.99650934988563,
3.10008230044163,3.20350555624704,3.30681221854458,3.41005628885965,3.51327152250986,
3.61649163431351,3.71982077793715,3.82320772460323,3.92677776279771,3.99534579984751,
4.09860814851249,4.20171513491833,4.30469859633615,4.40761536822811,4.51049968437655,
4.61338573414336,4.71637827780366,4.81942668398311,4.9226588076143,4.99418224980939,
5.09760357317468,5.20087154158791,5.30401821033476,5.40709947808644,5.51014934245976,
5.61320175788194,5.7163607823649,5.81957599567372,5.92297359909411,5.99301869977127,
6.09643423501026,6.19969678171232,6.30283860648639,6.40591538895671,6.50896113435575,
6.61200980509544,6.71516569207009,6.81837810297349,6.92177347981606,6.99185514973315,
7.09672279617372,7.20139614944408,7.2430409600995),.UNSPECIFIED.);
#901=B_SPLINE_CURVE_WITH_KNOTS('',3,(#89270,#89271,#89272,#89273,#89274,
#89275,#89276,#89277,#89278,#89279,#89280,#89281,#89282,#89283,#89284,#89285,
#89286,#89287,#89288,#89289,#89290,#89291,#89292,#89293,#89294,#89295),
 .UNSPECIFIED.,.F.,.F.,(4,2,2,2,2,2,2,2,2,2,2,2,4),(-0.0747573406682046,
-0.0739377203326066,-0.0616380686667433,-0.0559587372308882,-0.0377856382278336,
-0.0350634541223838,-0.0337175330335355,-0.0326484453300257,-0.0316335735595502,
-0.0303960837955203,-0.0285521200295371,-0.0215327131587606,-0.000655551428707696),
 .UNSPECIFIED.);
#902=B_SPLINE_CURVE_WITH_KNOTS('',3,(#89297,#89298,#89299,#89300,#89301,
#89302,#89303,#89304,#89305,#89306,#89307,#89308,#89309,#89310,#89311,#89312,
#89313,#89314,#89315,#89316,#89317,#89318,#89319,#89320,#89321,#89322,#89323,
#89324,#89325,#89326,#89327,#89328,#89329,#89330,#89331,#89332,#89333,#89334,
#89335,#89336,#89337,#89338,#89339,#89340,#89341,#89342,#89343,#89344,#89345,
#89346,#89347,#89348,#89349,#89350,#89351,#89352,#89353,#89354,#89355,#89356,
#89357,#89358,#89359,#89360,#89361,#89362,#89363,#89364,#89365,#89366,#89367,
#89368,#89369,#89370,#89371,#89372,#89373,#89374,#89375,#89376,#89377,#89378,
#89379,#89380,#89381,#89382,#89383,#89384,#89385,#89386,#89387,#89388,#89389,
#89390,#89391,#89392,#89393,#89394,#89395,#89396,#89397,#89398,#89399,#89400,
#89401,#89402,#89403,#89404,#89405,#89406,#89407,#89408,#89409,#89410,#89411,
#89412,#89413,#89414),.UNSPECIFIED.,.F.,.F.,(4,3,3,3,3,3,3,3,3,3,3,3,3,
3,3,3,3,3,3,3,3,3,3,3,3,3,3,3,3,3,3,3,3,3,3,3,3,3,3,4),(170.955339710339,
171.060905920727,171.162663398209,171.264353087631,171.366010720348,171.467671979169,
171.569433774406,171.671256095758,171.773239610404,171.799869393442,171.903390296067,
172.006760196182,172.110011759924,172.213199681674,172.316357783713,172.419519846812,
172.522789883762,172.626117040711,172.729626807232,172.798705843404,172.901009858667,
173.003159822786,173.105192383572,173.207162238204,173.309104751679,173.411055248523,
173.513128090537,173.615263928529,173.717605455249,173.797542293366,173.90381549814,
174.015385903789,174.121305781442,174.227126064404,174.332874494259,174.438578722884,
174.544296093967,174.650018553652,174.755813985758,174.796378743328),
 .UNSPECIFIED.);
#903=B_SPLINE_CURVE_WITH_KNOTS('',3,(#89418,#89419,#89420,#89421,#89422,
#89423,#89424,#89425,#89426,#89427,#89428,#89429,#89430,#89431,#89432,#89433,
#89434,#89435,#89436,#89437,#89438,#89439,#89440,#89441,#89442,#89443,#89444,
#89445,#89446,#89447,#89448,#89449,#89450,#89451,#89452,#89453,#89454,#89455,
#89456,#89457,#89458,#89459,#89460,#89461,#89462,#89463,#89464,#89465,#89466,
#89467,#89468,#89469,#89470,#89471,#89472,#89473,#89474,#89475,#89476,#89477,
#89478,#89479,#89480,#89481,#89482,#89483,#89484,#89485,#89486,#89487,#89488,
#89489,#89490,#89491,#89492,#89493,#89494,#89495,#89496,#89497,#89498,#89499,
#89500,#89501,#89502,#89503,#89504,#89505,#89506,#89507,#89508,#89509,#89510,
#89511,#89512,#89513,#89514,#89515,#89516,#89517,#89518,#89519,#89520,#89521,
#89522,#89523,#89524,#89525,#89526,#89527,#89528,#89529,#89530,#89531,#89532,
#89533,#89534,#89535,#89536,#89537,#89538,#89539,#89540,#89541,#89542,#89543,
#89544,#89545,#89546,#89547,#89548,#89549,#89550,#89551,#89552,#89553,#89554,
#89555,#89556,#89557,#89558,#89559,#89560,#89561,#89562,#89563,#89564,#89565,
#89566,#89567,#89568,#89569,#89570,#89571,#89572,#89573,#89574,#89575,#89576,
#89577,#89578,#89579,#89580,#89581,#89582,#89583,#89584,#89585,#89586),
 .UNSPECIFIED.,.F.,.F.,(4,3,3,3,3,3,3,3,3,3,3,3,3,3,3,3,3,3,3,3,3,3,3,3,
3,3,3,3,3,3,3,3,3,3,3,3,3,3,3,3,3,3,3,3,3,3,3,3,3,3,3,3,3,3,3,3,4),(-172.787594226707,
-172.684274547493,-172.581108276202,-172.478063417649,-172.375083759813,
-172.272135157488,-172.169183508487,-172.066127058214,-171.963013611671,
-171.859723903019,-171.799869393442,-171.696296383671,-171.592873066918,
-171.489566341367,-171.386322206412,-171.283106906827,-171.179886727883,
-171.076557515714,-170.973170499612,-170.8696003913,-170.80103294348,-170.697770746273,
-170.594663913509,-170.491680608289,-170.388763994098,-170.285879836938,
-170.182993947235,-170.08000156422,-169.976953319269,-169.873721356035,
-169.802196493519,-169.698775105051,-169.595507070885,-169.492360335737,
-169.38927900122,-169.286229069815,-169.183176587192,-169.080017495714,
-168.976802215422,-168.873404545781,-168.803360043557,-168.699944492337,
-168.59668192921,-168.493540087422,-168.390463287585,-168.287417524489,
-168.184368835746,-168.081212930417,-167.978000500935,-167.874605105352,
-167.804523593595,-167.699671782329,-167.594987983093,-167.490464931131,
-167.386036707514,-167.281667197445,-167.203857020092),.UNSPECIFIED.);
#904=B_SPLINE_CURVE_WITH_KNOTS('',3,(#89587,#89588,#89589,#89590,#89591,
#89592,#89593,#89594),.UNSPECIFIED.,.F.,.F.,(4,2,2,4),(-2.66749859469711,
-2.6454579420985,-2.59658607096104,-2.59330052944419),.UNSPECIFIED.);
#905=B_SPLINE_CURVE_WITH_KNOTS('',3,(#89599,#89600,#89601,#89602,#89603,
#89604,#89605,#89606,#89607,#89608,#89609,#89610,#89611,#89612,#89613,#89614,
#89615,#89616,#89617,#89618,#89619,#89620,#89621,#89622,#89623,#89624,#89625,
#89626,#89627,#89628,#89629,#89630,#89631,#89632,#89633,#89634,#89635,#89636,
#89637,#89638,#89639,#89640,#89641,#89642,#89643,#89644,#89645,#89646,#89647,
#89648,#89649,#89650,#89651,#89652,#89653,#89654,#89655,#89656,#89657,#89658,
#89659,#89660,#89661,#89662,#89663,#89664,#89665,#89666,#89667,#89668,#89669,
#89670,#89671,#89672,#89673,#89674,#89675,#89676,#89677,#89678,#89679,#89680,
#89681,#89682,#89683,#89684,#89685,#89686,#89687,#89688,#89689,#89690,#89691,
#89692,#89693,#89694,#89695,#89696,#89697,#89698,#89699,#89700,#89701,#89702,
#89703,#89704,#89705,#89706,#89707,#89708,#89709,#89710,#89711,#89712,#89713,
#89714,#89715,#89716,#89717,#89718,#89719,#89720,#89721,#89722,#89723,#89724,
#89725,#89726,#89727,#89728,#89729,#89730,#89731,#89732,#89733,#89734,#89735,
#89736,#89737,#89738,#89739,#89740,#89741,#89742,#89743,#89744,#89745,#89746,
#89747,#89748,#89749,#89750,#89751,#89752,#89753,#89754,#89755,#89756,#89757,
#89758,#89759,#89760,#89761,#89762,#89763,#89764,#89765,#89766,#89767,#89768,
#89769,#89770,#89771,#89772,#89773,#89774,#89775,#89776,#89777,#89778,#89779,
#89780,#89781,#89782,#89783,#89784,#89785,#89786,#89787,#89788,#89789,#89790,
#89791,#89792,#89793,#89794,#89795,#89796,#89797,#89798,#89799,#89800,#89801,
#89802,#89803,#89804,#89805,#89806,#89807,#89808,#89809,#89810,#89811,#89812,
#89813,#89814,#89815,#89816,#89817,#89818,#89819,#89820,#89821,#89822,#89823,
#89824),.UNSPECIFIED.,.F.,.F.,(4,2,2,2,2,2,2,2,2,2,2,2,2,2,2,2,2,2,2,2,
2,2,2,2,2,2,2,2,2,2,2,2,2,2,2,2,2,2,2,2,2,2,2,2,2,2,2,2,2,2,2,2,2,2,2,2,
2,2,2,2,2,2,2,2,2,2,2,2,2,2,2,2,2,2,2,2,2,2,2,2,2,2,2,2,2,2,2,2,2,2,2,2,
2,2,2,2,2,2,2,2,2,2,2,2,2,2,2,2,2,2,2,2,4),(-1.4081797897497,-1.40705404679594,
-1.40292854329057,-1.37574263320905,-1.33373204799533,-1.32763515619996,
-1.30978755234181,-1.30709916585643,-1.30573723651142,-1.30466495482482,
-1.30341928514225,-1.3011958614881,-1.29070305355408,-1.26784055652197,
-1.21011174840212,-1.20367847815884,-1.20117011677497,-1.19935225864924,
-1.19740896745055,-1.19480676077392,-1.18898303817082,-1.1651496956684,
-1.11614975325961,-1.09779133852374,-1.09505199725553,-1.09369780772592,
-1.09262570707542,-1.09137329073468,-1.08912119386837,-1.07817671240186,
-1.05366063720509,-0.998557317290027,-0.991850133661388,-0.989297520826545,
-0.98746765461196,-0.985529978993057,-0.982966721625732,-0.977358981402691,
-0.929074830132709,-0.888723629879558,-0.884011280685756,-0.882271307972931,
-0.881246023907791,-0.880154587919307,-0.878645291924542,-0.875062764192125,
-0.870037629013388,-0.856213724031729,-0.833863298665177,-0.787184837339988,
-0.779989343016949,-0.77707434241061,-0.775273826062298,-0.773322000949637,
-0.770660358982095,-0.764492288721172,-0.737949645692169,-0.698620518806667,
-0.687287343230985,-0.673503592179244,-0.671211207901103,-0.669826477407413,
-0.668750026953921,-0.667534893878322,-0.665449548519146,-0.656907908561592,
-0.64034708537071,-0.598277945699114,-0.571099480893947,-0.566971963994991,
-0.564479142149618,-0.562545400661154,-0.560449734724247,-0.557102213120062,
-0.545904425499174,-0.527329100099386,-0.484807662015825,-0.462028639108672,
-0.45917070499224,-0.457792035941198,-0.456715771265631,-0.455474801951997,
-0.453287245031174,-0.443435837807844,-0.394233153757333,-0.359839085039991,
-0.355551374847713,-0.353009378459771,-0.351065006828444,-0.348984721023599,
-0.345718697498416,-0.335297050035028,-0.318505517073179,-0.258883054465735,
-0.249294071881424,-0.247244741970683,-0.245918126656749,-0.244851087490946,
-0.243841364981986,-0.241868965805794,-0.234450932566741,-0.220917475641148,
-0.192337496364564,-0.147271544802984,-0.143024716885642,-0.140506642976319,
-0.138580632964851,-0.136520189151481,-0.133286020099834,-0.122977037585246,
-0.106384424931836,-0.0845184170571751,-0.0747573406682046),
 .UNSPECIFIED.);
#906=B_SPLINE_CURVE_WITH_KNOTS('',3,(#89825,#89826,#89827,#89828,#89829,
#89830,#89831,#89832,#89833,#89834,#89835,#89836,#89837,#89838,#89839,#89840,
#89841,#89842,#89843,#89844,#89845,#89846,#89847,#89848,#89849,#89850,#89851,
#89852,#89853,#89854,#89855,#89856,#89857,#89858,#89859,#89860,#89861,#89862,
#89863,#89864,#89865,#89866,#89867,#89868,#89869,#89870,#89871,#89872,#89873,
#89874,#89875,#89876,#89877,#89878,#89879,#89880,#89881,#89882,#89883,#89884,
#89885,#89886,#89887,#89888,#89889,#89890,#89891,#89892,#89893,#89894,#89895,
#89896,#89897,#89898,#89899,#89900,#89901,#89902,#89903,#89904,#89905,#89906,
#89907,#89908,#89909,#89910,#89911,#89912,#89913,#89914,#89915,#89916,#89917,
#89918,#89919,#89920,#89921,#89922,#89923,#89924,#89925,#89926,#89927,#89928,
#89929,#89930,#89931,#89932,#89933,#89934,#89935,#89936,#89937,#89938,#89939,
#89940,#89941,#89942,#89943,#89944,#89945,#89946,#89947,#89948,#89949,#89950,
#89951,#89952,#89953,#89954,#89955,#89956,#89957,#89958,#89959,#89960,#89961,
#89962,#89963,#89964,#89965,#89966,#89967,#89968,#89969,#89970,#89971,#89972,
#89973,#89974,#89975,#89976,#89977,#89978,#89979,#89980,#89981,#89982,#89983,
#89984,#89985,#89986,#89987,#89988,#89989,#89990,#89991,#89992,#89993,#89994,
#89995,#89996,#89997,#89998,#89999,#90000,#90001,#90002,#90003,#90004,#90005,
#90006,#90007,#90008,#90009,#90010,#90011,#90012,#90013,#90014,#90015,#90016,
#90017,#90018,#90019,#90020,#90021,#90022,#90023,#90024,#90025,#90026,#90027,
#90028,#90029,#90030,#90031,#90032,#90033,#90034,#90035,#90036,#90037,#90038,
#90039,#90040,#90041,#90042,#90043,#90044,#90045,#90046,#90047,#90048,#90049,
#90050,#90051,#90052,#90053,#90054,#90055,#90056),.UNSPECIFIED.,.F.,.F.,
(4,2,2,2,2,2,2,2,2,2,2,2,2,2,2,2,2,2,2,2,2,2,2,2,2,2,2,2,2,2,2,2,2,2,2,
2,2,2,2,2,2,2,2,2,2,2,2,2,2,2,2,2,2,2,2,2,2,2,2,2,2,2,2,2,2,2,2,2,2,2,2,
2,2,2,2,2,2,2,2,2,2,2,2,2,2,2,2,2,2,2,2,2,2,2,2,2,2,2,2,2,2,2,2,2,2,2,2,
2,2,2,2,2,2,2,2,4),(-2.59330052944419,-2.5868644382203,-2.58469323017153,
-2.5834597768618,-2.58238632325697,-2.58100820152467,-2.57814812648601,
-2.5420719383805,-2.50934246107363,-2.49296682459146,-2.48617192045704,
-2.48254547277301,-2.47944475000296,-2.4774380642021,-2.47549668507091,
-2.4729549099574,-2.46865955728029,-2.43366865647229,-2.38476726569877,
-2.37493625771775,-2.37275508398981,-2.37151813660649,-2.37044414131561,
-2.36906779445472,-2.3662171602355,-2.3298371603387,-2.2760372359654,-2.26958139117063,
-2.26686894554222,-2.26490655399863,-2.26311468811663,-2.2602539510892,
-2.25339519278051,-2.19997525375406,-2.17429633869993,-2.16304748871616,
-2.16077849703701,-2.15952290263944,-2.15845162975484,-2.1571031699405,
-2.15447767294023,-2.13831910533727,-2.09182445546661,-2.06385943680202,
-2.05751531889227,-2.05482203950276,-2.05286334176837,-2.05106781737619,
-2.04818587158402,-2.04119678880736,-1.98962010799096,-1.96265217495558,
-1.95107900283809,-1.94879167624671,-1.94753214900358,-1.94646113758936,
-1.94511764403119,-1.9425157239211,-1.92692673856165,-1.92044462760632,
-1.90654399156092,-1.8736598281375,-1.85710189143986,-1.84679336718953,
-1.84354474019463,-1.84147129836726,-1.839530385679,-1.83698873148448,-1.8326925176529,
-1.79749302106063,-1.74825035671139,-1.73886485807531,-1.73671544191209,
-1.73548585696091,-1.73441111209588,-1.73302459258726,-1.73012150501854,
-1.69805408790132,-1.66516506158529,-1.64633732657471,-1.63885274041799,
-1.63323030387704,-1.6306646562713,-1.62872695437746,-1.62689838542254,
-1.62434971995038,-1.61766602359586,-1.5622722677374,-1.53793035801725,
-1.52703149046051,-1.52478284395909,-1.52353153216006,-1.52245959751839,
-1.52110478414218,-1.51845058324905,-1.50156782970789,-1.48278043140398,
-1.44981441597523,-1.43316116010444,-1.42280939229993,-1.41955568845442,
-1.41748105804103,-1.41554047322765,-1.41300132605133,-1.40871400722063,
-1.36495318354359,-1.33390211915214,-1.3158515009014,-1.31315577159364,
-1.31179207184918,-1.31071940527398,-1.30947444268109,-1.30725504495263,
-1.29683145802611,-1.2742172493562,-1.25973288661493),.UNSPECIFIED.);
#907=B_SPLINE_CURVE_WITH_KNOTS('',3,(#90062,#90063,#90064,#90065),
 .UNSPECIFIED.,.F.,.F.,(4,4),(158.039785789401,158.388969095546),
 .UNSPECIFIED.);
#908=B_SPLINE_CURVE_WITH_KNOTS('',3,(#90066,#90067,#90068,#90069,#90070,
#90071,#90072,#90073,#90074,#90075,#90076,#90077,#90078,#90079,#90080,#90081,
#90082,#90083,#90084,#90085,#90086,#90087,#90088,#90089,#90090,#90091,#90092,
#90093,#90094,#90095,#90096,#90097,#90098,#90099,#90100,#90101,#90102,#90103,
#90104,#90105,#90106,#90107,#90108,#90109,#90110,#90111,#90112,#90113,#90114,
#90115,#90116,#90117,#90118,#90119,#90120,#90121,#90122,#90123,#90124,#90125,
#90126,#90127,#90128,#90129,#90130,#90131,#90132,#90133,#90134,#90135,#90136,
#90137,#90138,#90139,#90140,#90141,#90142,#90143,#90144,#90145,#90146,#90147,
#90148,#90149,#90150,#90151,#90152,#90153,#90154,#90155,#90156,#90157,#90158,
#90159,#90160,#90161,#90162,#90163,#90164,#90165,#90166,#90167,#90168,#90169,
#90170,#90171,#90172,#90173,#90174,#90175,#90176,#90177,#90178,#90179,#90180,
#90181,#90182,#90183,#90184,#90185,#90186,#90187,#90188,#90189,#90190,#90191,
#90192,#90193,#90194,#90195,#90196,#90197,#90198,#90199,#90200,#90201,#90202,
#90203,#90204,#90205,#90206,#90207,#90208,#90209,#90210,#90211,#90212,#90213,
#90214,#90215,#90216,#90217,#90218,#90219,#90220,#90221,#90222,#90223,#90224,
#90225,#90226,#90227,#90228,#90229,#90230,#90231,#90232,#90233,#90234,#90235,
#90236,#90237,#90238,#90239,#90240,#90241,#90242,#90243,#90244,#90245,#90246,
#90247,#90248,#90249,#90250,#90251,#90252,#90253,#90254,#90255,#90256,#90257,
#90258,#90259,#90260,#90261,#90262,#90263,#90264,#90265,#90266,#90267,#90268,
#90269,#90270,#90271,#90272,#90273,#90274,#90275),.UNSPECIFIED.,.F.,.F.,
(4,2,2,2,2,2,2,2,2,2,2,2,2,2,2,2,2,2,2,2,2,2,2,2,2,2,2,2,2,2,2,2,2,2,2,
2,2,2,2,2,2,2,2,2,2,2,2,2,2,2,2,2,2,2,2,2,2,2,2,2,2,2,2,2,2,2,2,2,2,2,2,
2,2,2,2,2,2,2,2,2,2,2,2,2,2,2,2,2,2,2,2,2,2,2,2,2,2,2,2,2,2,2,2,2,4),(-2.66742166532822,
-2.60891629431464,-2.59007759965161,-2.58078441649076,-2.57864191987016,
-2.57741400629466,-2.57633918293723,-2.57495056961282,-2.57203619767363,
-2.54225892562651,-2.49161776942559,-2.48229089683831,-2.47774055884935,
-2.47500299241396,-2.47251919503927,-2.4706432007799,-2.46881661986733,
-2.4662747913464,-2.45963351799724,-2.40385355530975,-2.37977593050351,
-2.36894872217324,-2.36670461920435,-2.36545440107624,-2.36438251077472,
-2.36302660964724,-2.36088140526517,-2.34984929619756,-2.29862561393848,
-2.26992229051696,-2.26348941257987,-2.2607809377382,-2.25881936010741,
-2.25702682155979,-2.25416193435291,-2.24727728246947,-2.19421613294384,
-2.16830170531865,-2.15699288850901,-2.15472039428576,-2.15346401275327,
-2.15239274193152,-2.15104514151731,-2.14842389176343,-2.1323854468327,
-2.12706553014289,-2.11250729619373,-2.07961705160713,-2.06305105501089,
-2.052739197494,-2.04949042823377,-2.0474171168656,-2.04547648279748,-2.04293542081362,
-2.03864072394683,-2.00353402401563,-1.95464777307175,-1.94485963447044,
-1.94268230549169,-1.94144668958548,-1.94037300444971,-1.93899617558637,
-1.93614233737396,-1.91342989016208,-1.87271609682472,-1.84567950042459,
-1.83944815818842,-1.83677392874418,-1.83481835251845,-1.83301820237483,
-1.83011227275717,-1.82298113247133,-1.7742477543539,-1.73505282196107,
-1.73147807388371,-1.72996904762295,-1.72887688066177,-1.72785089843548,
-1.72610770396323,-1.7213747511041,-1.68178083770795,-1.63388986142474,
-1.6274930935136,-1.62479052386571,-1.62282983325471,-1.62103576815868,
-1.61816334456911,-1.61123416775846,-1.55875577244843,-1.53242881078123,
-1.52101504710523,-1.518736408709,-1.51747862427611,-1.5164074510596,-1.5150615897315,
-1.51244824985317,-1.49656852752491,-1.49069764502866,-1.44666704061987,
-1.42810816395616,-1.41691845749845,-1.41357286260411,-1.41147833591662,
-1.40954560786303,-1.4081797897497),.UNSPECIFIED.);
#909=B_SPLINE_CURVE_WITH_KNOTS('',3,(#90277,#90278,#90279,#90280,#90281,
#90282,#90283,#90284,#90285,#90286,#90287,#90288,#90289,#90290,#90291,#90292,
#90293,#90294,#90295,#90296,#90297,#90298,#90299,#90300,#90301,#90302,#90303,
#90304,#90305,#90306,#90307,#90308,#90309,#90310,#90311,#90312,#90313,#90314,
#90315,#90316,#90317,#90318,#90319,#90320,#90321,#90322,#90323,#90324,#90325,
#90326,#90327,#90328,#90329,#90330,#90331,#90332,#90333,#90334,#90335,#90336,
#90337,#90338,#90339,#90340,#90341,#90342,#90343,#90344,#90345,#90346,#90347,
#90348,#90349,#90350,#90351,#90352,#90353,#90354,#90355,#90356,#90357,#90358,
#90359,#90360,#90361,#90362,#90363,#90364,#90365,#90366,#90367,#90368,#90369,
#90370,#90371,#90372,#90373,#90374,#90375,#90376,#90377,#90378,#90379,#90380,
#90381,#90382,#90383,#90384,#90385,#90386,#90387,#90388,#90389,#90390,#90391,
#90392,#90393,#90394,#90395,#90396,#90397,#90398,#90399,#90400,#90401,#90402,
#90403,#90404,#90405,#90406,#90407,#90408,#90409,#90410,#90411,#90412,#90413,
#90414,#90415,#90416,#90417,#90418,#90419,#90420,#90421,#90422,#90423,#90424,
#90425,#90426,#90427,#90428,#90429,#90430,#90431,#90432,#90433,#90434,#90435,
#90436,#90437,#90438,#90439,#90440,#90441,#90442,#90443,#90444,#90445,#90446,
#90447,#90448,#90449,#90450,#90451,#90452,#90453,#90454,#90455,#90456,#90457,
#90458,#90459,#90460,#90461,#90462,#90463,#90464,#90465,#90466,#90467,#90468,
#90469,#90470,#90471,#90472,#90473,#90474,#90475,#90476,#90477,#90478,#90479,
#90480,#90481,#90482,#90483,#90484,#90485,#90486,#90487,#90488,#90489,#90490,
#90491,#90492,#90493,#90494),.UNSPECIFIED.,.F.,.F.,(4,2,2,2,2,2,2,2,2,2,
2,2,2,2,2,2,2,2,2,2,2,2,2,2,2,2,2,2,2,2,2,2,2,2,2,2,2,2,2,2,2,2,2,2,2,2,
2,2,2,2,2,2,2,2,2,2,2,2,2,2,2,2,2,2,2,2,2,2,2,2,2,2,2,2,2,2,2,2,2,2,2,2,
2,2,2,2,2,2,2,2,2,2,2,2,2,2,2,2,2,2,2,2,2,2,2,2,2,2,4),(-1.25973288661493,
-1.21609102900778,-1.20970713987316,-1.20720678920522,-1.20539086341582,
-1.2034460086005,-1.20083540243935,-1.19496613525091,-1.17078874386512,
-1.12030360124663,-1.1198718858852,-1.10368544639769,-1.10105841432207,
-1.09970942323476,-1.09863788976092,-1.09738218819883,-1.09511335897906,
-1.08387288766232,-1.05822562808826,-1.00472263010325,-0.997868278970091,
-0.995008121823537,-0.993216256726692,-0.991253580237683,-0.988540206969882,
-0.982079601166141,-0.928143971185043,-0.891931386762398,-0.889076756241666,
-0.887699689127835,-0.886625881524295,-0.885390202485962,-0.883212937621884,
-0.873428338083152,-0.82450744678719,-0.789384468975772,-0.78508906511928,
-0.782547717715193,-0.780606931002825,-0.778533518822625,-0.775284719997248,
-0.764973758756719,-0.748412426730895,-0.715552856294598,-0.701808196570598,
-0.694966711579718,-0.694678201475862,-0.689570275476756,-0.679120560118283,
-0.677012539820711,-0.675667992911381,-0.674596860609576,-0.673337992108514,
-0.671054196041308,-0.65954849637835,-0.632851307566126,-0.580856958608613,
-0.573892440975401,-0.571014328735491,-0.56921933296634,-0.567259729978056,
-0.564562494512965,-0.558196344731607,-0.530055119346326,-0.482629510166844,
-0.476764228666177,-0.4670299106766,-0.464970429658426,-0.463640820803762,
-0.462570511786875,-0.461299580938961,-0.458959845461074,-0.446402754509434,
-0.388606908516483,-0.381963461977945,-0.364258386221868,-0.360585764722962,
-0.358204522639127,-0.356289599767679,-0.354110024598494,-0.350380157895714,
-0.334899452064879,-0.283061726071859,-0.256023268574076,-0.253121793407635,
-0.251735740873461,-0.250661241279027,-0.249431849008249,-0.247325610837725,
-0.238412497268297,-0.220688901717591,-0.192467064558443,-0.153492447207531,
-0.14875578850538,-0.146329879720163,-0.144410718331475,-0.142259821620451,
-0.138659930148412,-0.124800709222653,-0.0975397305688386,-0.0749682922101801,
-0.0441240160777874,-0.0412117837959577,-0.0398236655310865,-0.0387489802648021,
-0.0375209594861392,-0.0362288352709404,-0.0342508952684674,-0.000628703082161277),
 .UNSPECIFIED.);
#910=B_SPLINE_CURVE_WITH_KNOTS('',3,(#90495,#90496,#90497,#90498,#90499,
#90500,#90501,#90502,#90503,#90504,#90505,#90506,#90507,#90508,#90509,#90510,
#90511,#90512),.UNSPECIFIED.,.F.,.F.,(4,2,2,2,2,2,2,2,4),(-2.66821958497409,
-2.63796945984048,-2.61126613950847,-2.60507567789451,-2.6024083434344,
-2.60045381523792,-2.59865183150659,-2.59573671182581,-2.59373671315012),
 .UNSPECIFIED.);
#911=B_SPLINE_CURVE_WITH_KNOTS('',3,(#90518,#90519,#90520,#90521,#90522,
#90523,#90524,#90525,#90526,#90527,#90528,#90529,#90530),.UNSPECIFIED.,
 .F.,.F.,(4,3,3,3,4),(151.755345396259,151.823140394205,151.95194859726,
152.078650414049,152.105783788367),.UNSPECIFIED.);
#912=B_SPLINE_CURVE_WITH_KNOTS('',3,(#90531,#90532,#90533,#90534,#90535,
#90536,#90537,#90538,#90539,#90540),.UNSPECIFIED.,.F.,.F.,(4,1,1,1,1,1,
1,4),(152.105783788367,152.821976844167,153.820813294129,154.81964974409,
155.818486194052,156.817322644014,157.816159093976,158.039785789401),
 .UNSPECIFIED.);
#913=B_SPLINE_CURVE_WITH_KNOTS('',3,(#90541,#90542,#90543,#90544,#90545,
#90546,#90547,#90548,#90549,#90550,#90551,#90552,#90553,#90554,#90555,#90556,
#90557,#90558,#90559,#90560,#90561,#90562,#90563,#90564,#90565,#90566,#90567,
#90568,#90569,#90570,#90571,#90572,#90573,#90574,#90575,#90576,#90577,#90578,
#90579,#90580,#90581,#90582,#90583,#90584,#90585,#90586,#90587,#90588,#90589,
#90590,#90591,#90592,#90593,#90594,#90595,#90596,#90597,#90598,#90599,#90600,
#90601,#90602,#90603,#90604,#90605,#90606,#90607,#90608,#90609,#90610,#90611,
#90612,#90613,#90614,#90615,#90616,#90617,#90618,#90619,#90620,#90621,#90622,
#90623,#90624,#90625,#90626,#90627,#90628,#90629,#90630,#90631,#90632,#90633,
#90634,#90635,#90636,#90637,#90638,#90639,#90640,#90641,#90642,#90643,#90644,
#90645,#90646,#90647,#90648,#90649,#90650,#90651,#90652,#90653,#90654,#90655,
#90656,#90657,#90658,#90659,#90660,#90661,#90662,#90663,#90664,#90665,#90666,
#90667,#90668,#90669,#90670,#90671,#90672,#90673,#90674,#90675,#90676,#90677,
#90678,#90679,#90680,#90681,#90682,#90683,#90684,#90685,#90686,#90687,#90688,
#90689,#90690,#90691,#90692,#90693,#90694,#90695,#90696,#90697,#90698,#90699,
#90700,#90701,#90702,#90703,#90704,#90705,#90706,#90707,#90708,#90709,#90710,
#90711,#90712,#90713,#90714,#90715,#90716,#90717,#90718,#90719,#90720,#90721,
#90722,#90723,#90724,#90725,#90726,#90727,#90728,#90729,#90730,#90731,#90732,
#90733,#90734,#90735,#90736,#90737,#90738,#90739,#90740,#90741,#90742,#90743,
#90744,#90745,#90746,#90747,#90748,#90749,#90750,#90751,#90752,#90753,#90754,
#90755,#90756,#90757,#90758,#90759,#90760,#90761,#90762),.UNSPECIFIED.,
 .F.,.F.,(4,2,2,2,2,2,2,2,2,2,2,2,2,2,2,2,2,2,2,2,2,2,2,2,2,2,2,2,2,2,2,
2,2,2,2,2,2,2,2,2,2,2,2,2,2,2,2,2,2,2,2,2,2,2,2,2,2,2,2,2,2,2,2,2,2,2,2,
2,2,2,2,2,2,2,2,2,2,2,2,2,2,2,2,2,2,2,2,2,2,2,2,2,2,2,2,2,2,2,2,2,2,2,2,
2,2,2,2,2,2,2,4),(-2.59373671315012,-2.5885519066095,-2.54144355714508,
-2.51722412424279,-2.5050149229938,-2.49811631989247,-2.49617311223199,
-2.49515834494911,-2.49408693164924,-2.49274001307796,-2.4901226509639,
-2.47415863689511,-2.46978685897904,-2.42630149968854,-2.39931492302155,
-2.3930894522106,-2.39041606572864,-2.38846047946461,-2.3866598821561,-2.38375225793744,
-2.37661209459938,-2.32808667121904,-2.28870985303142,-2.28511725563706,
-2.28360510789293,-2.28251234203669,-2.28148717219389,-2.27974816493781,
-2.2750429161707,-2.23449993456854,-2.18634894413985,-2.1807425250122,-2.17817981629052,
-2.17624254297965,-2.1744130567236,-2.17186098219802,-2.16515526905852,
-2.10999239957505,-2.08549800701937,-2.07455840148644,-2.07230726977264,
-2.07105539593064,-2.06998348286275,-2.06862933946845,-2.06589031332082,
-2.0475474466011,-2.02964507883391,-1.99690756912366,-1.97439761841213,
-1.96875036813469,-1.9661799996026,-1.96424142342186,-1.96241400913326,
-1.95987013454753,-1.95321821753177,-1.89749321116305,-1.87336612025167,
-1.86252449021087,-1.86027911629667,-1.8590284306805,-1.85795629518206,
-1.85660028092841,-1.85445525614602,-1.84343170659804,-1.79212690887746,
-1.76346286191477,-1.75703392161832,-1.75432571791138,-1.75236383347144,
-1.7505706684644,-1.74770402737221,-1.74081126317658,-1.68781786469749,
-1.66184078828374,-1.65051483902675,-1.64824095990395,-1.64698408922861,
-1.64591255628575,-1.64456482815435,-1.6419439561885,-1.62591896321951,
-1.62051407716177,-1.60601449268855,-1.57311679546957,-1.55035891717881,
-1.5446779925067,-1.54210133553019,-1.54016168247121,-1.53833594190101,
-1.53579870545865,-1.52918963838033,-1.47303657279827,-1.44918592382808,
-1.43841875724763,-1.4361777985978,-1.43492802304568,-1.4338557112365,-1.43249824599391,
-1.42983233030584,-1.41264466940409,-1.36256430977398,-1.34500777813006,
-1.33425295364739,-1.33095371188329,-1.32886892153168,-1.32693190827543,
-1.32437257649212,-1.3187857356506,-1.31136194166418,-1.29275925442224,
-1.25991250331722),.UNSPECIFIED.);
#914=B_SPLINE_CURVE_WITH_KNOTS('',3,(#90768,#90769,#90770,#90771,#90772,
#90773,#90774,#90775,#90776,#90777,#90778,#90779,#90780,#90781),
 .UNSPECIFIED.,.F.,.F.,(4,2,2,2,2,2,4),(-0.074917573155471,-0.0721518777810642,
-0.0417414976932024,-0.00539305516346449,-0.00193455376436665,-0.000863977439296385,
-0.000629063808748724),.UNSPECIFIED.);
#915=B_SPLINE_CURVE_WITH_KNOTS('',3,(#90782,#90783,#90784,#90785,#90786,
#90787,#90788,#90789,#90790,#90791,#90792,#90793,#90794,#90795,#90796,#90797,
#90798,#90799,#90800,#90801,#90802,#90803,#90804,#90805,#90806,#90807,#90808,
#90809,#90810,#90811,#90812,#90813,#90814,#90815,#90816,#90817,#90818,#90819,
#90820,#90821,#90822,#90823,#90824,#90825,#90826,#90827,#90828,#90829,#90830,
#90831,#90832,#90833,#90834,#90835,#90836,#90837,#90838,#90839,#90840,#90841,
#90842,#90843,#90844,#90845,#90846,#90847,#90848,#90849,#90850,#90851,#90852,
#90853,#90854,#90855,#90856,#90857,#90858,#90859,#90860,#90861,#90862,#90863,
#90864,#90865,#90866,#90867,#90868,#90869,#90870,#90871,#90872,#90873,#90874,
#90875,#90876,#90877,#90878,#90879,#90880,#90881,#90882,#90883,#90884,#90885,
#90886,#90887,#90888,#90889,#90890,#90891,#90892,#90893,#90894,#90895,#90896,
#90897,#90898,#90899,#90900,#90901,#90902,#90903,#90904,#90905,#90906,#90907,
#90908,#90909,#90910,#90911,#90912,#90913,#90914,#90915,#90916,#90917,#90918,
#90919,#90920,#90921,#90922,#90923,#90924,#90925,#90926,#90927,#90928,#90929,
#90930,#90931,#90932,#90933,#90934,#90935,#90936,#90937,#90938,#90939,#90940,
#90941,#90942,#90943,#90944,#90945,#90946,#90947,#90948,#90949,#90950,#90951,
#90952,#90953,#90954,#90955,#90956,#90957,#90958,#90959,#90960,#90961,#90962),
 .UNSPECIFIED.,.F.,.F.,(4,3,3,3,3,3,3,3,3,3,3,3,3,3,3,3,3,3,3,3,3,3,3,3,
3,3,3,3,3,3,3,3,3,3,3,3,3,3,3,3,3,3,3,3,3,3,3,3,3,3,3,3,3,3,3,3,3,3,3,3,
4),(145.822598481187,145.830121694434,145.93351643147,146.036757713573,
146.139877678953,146.24293224715,146.345955455496,146.448981298156,146.552114064923,
146.655303156322,146.758675149692,146.828958144396,146.932352881429,147.03559416353,
147.138714128907,147.241768697101,147.344791905443,147.4478177481,147.550950514863,
147.654139606258,147.757511599624,147.827794594357,147.931189331481,148.034430613671,
148.137550579139,148.240605147424,148.343628355857,148.446654198605,148.549786965457,
148.652976056941,148.756348050394,148.826631044319,148.930025781262,149.033267063273,
149.136387028563,149.239441596669,149.342464804925,149.445490647497,149.548623414176,
149.651812505488,149.755184498775,149.825467494281,149.928862231266,150.032103513317,
150.135223478643,150.238278046785,150.341301255075,150.444327097679,150.547459864388,
150.650648955728,150.75402094904,150.824303944243,150.927703487107,151.031158725751,
151.134277032305,151.237328082822,151.340345915983,151.444095786052,151.547200179005,
151.651272787632,151.755345396259),.UNSPECIFIED.);
#916=B_SPLINE_CURVE_WITH_KNOTS('',3,(#90964,#90965,#90966,#90967,#90968,
#90969,#90970,#90971,#90972,#90973,#90974,#90975,#90976,#90977,#90978,#90979,
#90980,#90981,#90982,#90983,#90984,#90985,#90986,#90987,#90988,#90989,#90990,
#90991,#90992,#90993,#90994,#90995,#90996,#90997,#90998,#90999,#91000,#91001,
#91002,#91003,#91004,#91005,#91006,#91007,#91008,#91009,#91010,#91011,#91012,
#91013,#91014,#91015,#91016,#91017,#91018,#91019,#91020,#91021,#91022,#91023,
#91024,#91025,#91026,#91027,#91028,#91029,#91030,#91031,#91032,#91033,#91034,
#91035,#91036,#91037,#91038,#91039,#91040,#91041,#91042,#91043,#91044,#91045,
#91046,#91047,#91048,#91049,#91050,#91051,#91052,#91053,#91054,#91055,#91056,
#91057,#91058,#91059,#91060,#91061,#91062,#91063,#91064,#91065,#91066,#91067,
#91068,#91069,#91070,#91071,#91072,#91073,#91074,#91075,#91076,#91077,#91078,
#91079,#91080,#91081,#91082,#91083,#91084,#91085,#91086,#91087,#91088,#91089,
#91090,#91091,#91092,#91093,#91094,#91095,#91096,#91097,#91098,#91099,#91100,
#91101,#91102,#91103,#91104,#91105,#91106,#91107,#91108,#91109,#91110,#91111,
#91112,#91113,#91114,#91115,#91116,#91117,#91118,#91119,#91120,#91121,#91122,
#91123,#91124,#91125,#91126,#91127,#91128,#91129,#91130,#91131,#91132,#91133,
#91134,#91135,#91136,#91137,#91138,#91139,#91140,#91141,#91142,#91143,#91144,
#91145,#91146,#91147,#91148,#91149,#91150,#91151,#91152,#91153,#91154,#91155,
#91156,#91157,#91158,#91159,#91160,#91161,#91162,#91163,#91164,#91165,#91166,
#91167,#91168,#91169,#91170,#91171,#91172,#91173,#91174,#91175,#91176,#91177,
#91178,#91179,#91180,#91181,#91182,#91183,#91184,#91185,#91186,#91187),
 .UNSPECIFIED.,.F.,.F.,(4,2,2,2,2,2,2,2,2,2,2,2,2,2,2,2,2,2,2,2,2,2,2,2,
2,2,2,2,2,2,2,2,2,2,2,2,2,2,2,2,2,2,2,2,2,2,2,2,2,2,2,2,2,2,2,2,2,2,2,2,
2,2,2,2,2,2,2,2,2,2,2,2,2,2,2,2,2,2,2,2,2,2,2,2,2,2,2,2,2,2,2,2,2,2,2,2,
2,2,2,2,2,2,2,2,2,2,2,2,2,2,2,4),(-1.25991250331722,-1.25002813172122,-1.22739940627457,
-1.22454711829876,-1.22317040286594,-1.22209650344233,-1.22086030515237,
-1.2186811330972,-1.20887147997461,-1.15996413031623,-1.12484337567231,
-1.12054749914052,-1.11800584391394,-1.11606480586091,-1.1139911093724,
-1.11074183203824,-1.10042907261466,-1.0838645839366,-1.05099990909305,
-1.03717125190871,-1.03052074071258,-1.01504656714291,-1.01244937440331,
-1.01110681137823,-1.0100356707126,-1.0087749432634,-1.00648302703673,-0.994835746195091,
-0.967567893194984,-0.947382757239736,-0.912873674362607,-0.908586806373821,
-0.906047786917541,-0.904107208166566,-0.902032494225878,-0.898778469395456,
-0.888423975695388,-0.871767003261979,-0.838826047861659,-0.820097788600979,
-0.803187225981111,-0.800532039099481,-0.799177010426617,-0.798105054208289,
-0.796853893602148,-0.794605944819627,-0.783719158342336,-0.759419477194735,
-0.703923634882994,-0.697247249399042,-0.694699731403431,-0.692871485664991,
-0.690933666987531,-0.688367078274858,-0.682739383699102,-0.6752465152499,
-0.656390000490043,-0.626123162780596,-0.603712281586419,-0.590881821532613,
-0.588635417285089,-0.587248847445616,-0.586174186400526,-0.584944877850398,
-0.582796222107857,-0.573418765837406,-0.524153447857989,-0.488926995616057,
-0.484630621662475,-0.482089118915688,-0.480148454556145,-0.478075406677634,
-0.474827666243869,-0.464524171507818,-0.447978733805499,-0.417105330677107,
-0.397465074860393,-0.379318159348492,-0.376619772926513,-0.375255700043835,
-0.374183243301061,-0.37293910482788,-0.370722563288281,-0.360689042936503,
-0.312017030045687,-0.276983409152321,-0.272689986985027,-0.270149477771124,
-0.268209138599189,-0.266136017776191,-0.262887285387177,-0.252768494669576,
-0.236546077612513,-0.198322587460796,-0.167652355216197,-0.164739955529095,
-0.163351845156246,-0.16227720647158,-0.161049284316136,-0.159757277992429,
-0.155110106732141,-0.128864893842154,-0.106990886444038,-0.105560222755592,
-0.0651104975484208,-0.0603738601673643,-0.0579480736817614,-0.0560290637262798,
-0.0538783940734142,-0.0516516914803666,-0.0483298719004753,-0.0006289855317579),
 .UNSPECIFIED.);
#917=B_SPLINE_CURVE_WITH_KNOTS('',3,(#91188,#91189,#91190,#91191,#91192,
#91193,#91194,#91195,#91196,#91197,#91198,#91199,#91200,#91201,#91202,#91203,
#91204,#91205,#91206,#91207),.UNSPECIFIED.,.F.,.F.,(4,2,2,2,2,2,2,2,2,4),
(-2.66776155019002,-2.62480392487054,-2.62186972745952,-2.62018685021,-2.61868180779369,
-2.61759012196051,-2.61656272724315,-2.61481300241367,-2.61003839935785,
-2.59362782388558),.UNSPECIFIED.);
#918=B_SPLINE_CURVE_WITH_KNOTS('',3,(#91212,#91213,#91214,#91215,#91216,
#91217,#91218,#91219,#91220,#91221,#91222,#91223,#91224,#91225,#91226,#91227,
#91228,#91229,#91230,#91231,#91232,#91233,#91234,#91235,#91236,#91237,#91238,
#91239,#91240,#91241,#91242,#91243,#91244,#91245,#91246,#91247,#91248,#91249,
#91250,#91251,#91252,#91253,#91254,#91255,#91256,#91257,#91258,#91259,#91260,
#91261,#91262,#91263,#91264,#91265,#91266,#91267,#91268,#91269,#91270,#91271,
#91272,#91273,#91274,#91275,#91276,#91277,#91278,#91279,#91280,#91281,#91282,
#91283,#91284,#91285,#91286,#91287,#91288,#91289,#91290,#91291,#91292,#91293,
#91294,#91295,#91296,#91297,#91298,#91299,#91300,#91301,#91302,#91303,#91304,
#91305,#91306,#91307,#91308,#91309,#91310,#91311,#91312,#91313,#91314,#91315,
#91316,#91317,#91318,#91319,#91320,#91321,#91322,#91323,#91324,#91325,#91326,
#91327,#91328,#91329,#91330,#91331,#91332,#91333,#91334,#91335,#91336,#91337,
#91338,#91339,#91340,#91341,#91342,#91343,#91344,#91345,#91346,#91347,#91348,
#91349,#91350,#91351,#91352,#91353,#91354,#91355,#91356,#91357,#91358,#91359,
#91360,#91361,#91362,#91363,#91364,#91365,#91366,#91367,#91368,#91369,#91370,
#91371,#91372,#91373,#91374,#91375,#91376,#91377,#91378,#91379,#91380,#91381,
#91382,#91383,#91384,#91385,#91386,#91387,#91388,#91389,#91390,#91391,#91392,
#91393,#91394,#91395,#91396,#91397,#91398,#91399,#91400,#91401,#91402,#91403,
#91404,#91405,#91406,#91407,#91408,#91409,#91410,#91411,#91412,#91413,#91414,
#91415,#91416,#91417,#91418,#91419,#91420,#91421,#91422,#91423,#91424,#91425,
#91426,#91427,#91428,#91429,#91430,#91431,#91432,#91433,#91434,#91435,#91436,
#91437,#91438,#91439,#91440,#91441,#91442,#91443,#91444,#91445,#91446,#91447,
#91448,#91449,#91450,#91451,#91452,#91453,#91454,#91455,#91456,#91457,#91458,
#91459,#91460,#91461,#91462,#91463,#91464,#91465,#91466,#91467,#91468,#91469,
#91470,#91471,#91472,#91473,#91474,#91475,#91476,#91477,#91478,#91479,#91480,
#91481,#91482,#91483,#91484,#91485,#91486,#91487,#91488,#91489,#91490,#91491,
#91492,#91493,#91494,#91495,#91496,#91497,#91498,#91499,#91500,#91501,#91502,
#91503),.UNSPECIFIED.,.F.,.F.,(4,2,2,2,2,2,2,2,2,2,2,2,2,2,2,2,2,2,2,2,
2,2,2,2,2,2,2,2,2,2,2,2,2,2,2,2,2,2,2,2,2,2,2,2,2,2,2,2,2,2,2,2,2,2,2,2,
2,2,2,2,2,2,2,2,2,2,2,2,2,2,2,2,2,2,2,2,2,2,2,2,2,2,2,2,2,2,2,2,2,2,2,2,
2,2,2,2,2,2,2,2,2,2,2,2,2,2,2,2,2,2,2,2,2,2,2,2,2,2,2,2,2,2,2,2,2,2,2,2,
2,2,2,2,2,2,2,2,2,2,2,2,2,2,2,2,2,4),(-1.40850263276381,-1.39306960650067,
-1.38272141396964,-1.37946833818062,-1.37739398881794,-1.37545358293386,
-1.37291454863777,-1.36862714823561,-1.33404430226293,-1.27807589774523,
-1.27380186776896,-1.2721302118413,-1.27111813467408,-1.27001574616159,
-1.26845075233166,-1.26453804111152,-1.24532482158701,-1.18894817501761,
-1.17210239448734,-1.16848552089998,-1.16612131436722,-1.16420743009777,
-1.16201517432855,-1.15822869517727,-1.14198122170515,-1.08450354925769,
-1.07953139272385,-1.06354559320653,-1.06092713862079,-1.05958002512239,
-1.05850864967895,-1.05725158550547,-1.05497638394429,-1.04362442710341,
-1.01754024734705,-0.964668867744824,-0.957765554845653,-0.954897388799684,
-0.953104103693257,-0.951142763526614,-0.94843654163411,-0.942018110998607,
-0.913442873113261,-0.862247029074522,-0.85108306084867,-0.848929648340678,
-0.847571185754394,-0.846499019082565,-0.845250490378984,-0.843014434882705,
-0.832321750132846,-0.808737936343438,-0.752153096626779,-0.74558954398186,
-0.743059903887193,-0.741236436515012,-0.739296246194381,-0.73671381893069,
-0.730999356023087,-0.707989940413683,-0.674964337528586,-0.653790273629086,
-0.639415317281718,-0.637089629359933,-0.635694469611654,-0.634616103399286,
-0.633406012254734,-0.631343979448014,-0.623093436484699,-0.60736981153309,
-0.565372529404616,-0.537089951379794,-0.532935397739698,-0.530435236908605,
-0.528501113236433,-0.526410322838754,-0.523082025283081,-0.512054952853508,
-0.493875879415992,-0.444530095327261,-0.427621884538517,-0.424967090879969,
-0.423612265100394,-0.422540470539185,-0.421289499927994,-0.41904189577949,
-0.408156841471152,-0.383861158966252,-0.328373211450144,-0.321697882679927,
-0.319150756769556,-0.317322788963908,-0.315385261708537,-0.312819053600094,
-0.3071921717625,-0.299700372490152,-0.280846477358196,-0.243379611800286,
-0.215989461150098,-0.213146930991104,-0.2117665626231,-0.210714902543605,
-0.210704908166831,-0.210695219542147,-0.210685813785961,-0.210676670313867,
-0.210667770546727,-0.210659097713162,-0.210650636523358,-0.210642372995015,
-0.210634294452222,-0.210626389153954,-0.210618646320887,-0.21061105611836,
-0.210603609337558,-0.210596297508208,-0.210589112793029,-0.210582047896446,
-0.210575095924169,-0.210568250483994,-0.210561505639592,-0.21055485581026,
-0.210548295784861,-0.210541820529687,-0.21053542544248,-0.210529106212553,
-0.210522858613384,-0.210516678751372,-0.210510562912216,-0.210504507472682,
-0.21049850917729,-0.210492564804552,-0.210486671239849,-0.210480825664762,
-0.209218777563569,-0.206836330089074,-0.193388474596719,-0.157804786601052,
-0.113366713485948,-0.109089406061395,-0.106553552524982,-0.104613951666928,
-0.102538881528046,-0.0992813619648698,-0.0888907940615931,-0.074917573155471),
 .UNSPECIFIED.);
#919=B_SPLINE_CURVE_WITH_KNOTS('',3,(#91504,#91505,#91506,#91507,#91508,
#91509,#91510,#91511,#91512,#91513,#91514,#91515,#91516,#91517,#91518,#91519,
#91520,#91521,#91522,#91523,#91524,#91525,#91526,#91527,#91528,#91529,#91530,
#91531,#91532,#91533,#91534,#91535,#91536,#91537,#91538,#91539,#91540,#91541,
#91542,#91543,#91544,#91545,#91546,#91547,#91548,#91549,#91550,#91551,#91552,
#91553,#91554,#91555,#91556,#91557,#91558,#91559,#91560,#91561,#91562,#91563,
#91564,#91565,#91566,#91567,#91568,#91569,#91570,#91571,#91572,#91573,#91574,
#91575,#91576,#91577,#91578,#91579,#91580,#91581,#91582,#91583,#91584,#91585,
#91586,#91587,#91588,#91589,#91590,#91591,#91592,#91593,#91594,#91595,#91596,
#91597,#91598,#91599,#91600,#91601,#91602,#91603,#91604,#91605,#91606,#91607,
#91608,#91609,#91610,#91611,#91612,#91613,#91614,#91615,#91616,#91617,#91618,
#91619,#91620,#91621,#91622,#91623,#91624,#91625,#91626,#91627,#91628,#91629,
#91630,#91631,#91632,#91633,#91634,#91635,#91636,#91637,#91638,#91639,#91640,
#91641,#91642,#91643,#91644,#91645,#91646,#91647,#91648,#91649,#91650,#91651,
#91652,#91653,#91654,#91655,#91656,#91657,#91658,#91659,#91660,#91661,#91662,
#91663,#91664,#91665,#91666,#91667,#91668,#91669,#91670,#91671,#91672,#91673,
#91674,#91675,#91676,#91677,#91678,#91679,#91680,#91681,#91682,#91683,#91684,
#91685,#91686,#91687,#91688,#91689,#91690,#91691,#91692,#91693,#91694,#91695,
#91696,#91697,#91698,#91699,#91700,#91701,#91702,#91703,#91704,#91705,#91706,
#91707,#91708,#91709,#91710,#91711,#91712,#91713,#91714,#91715,#91716,#91717,
#91718,#91719,#91720,#91721,#91722,#91723,#91724,#91725,#91726,#91727,#91728,
#91729),.UNSPECIFIED.,.F.,.F.,(4,2,2,2,2,2,2,2,2,2,2,2,2,2,2,2,2,2,2,2,
2,2,2,2,2,2,2,2,2,2,2,2,2,2,2,2,2,2,2,2,2,2,2,2,2,2,2,2,2,2,2,2,2,2,2,2,
2,2,2,2,2,2,2,2,2,2,2,2,2,2,2,2,2,2,2,2,2,2,2,2,2,2,2,2,2,2,2,2,2,2,2,2,
2,2,2,2,2,2,2,2,2,2,2,2,2,2,2,2,2,2,2,2,4),(-2.59362782388558,-2.57257925030196,
-2.55115577851568,-2.5228183915866,-2.51634429103098,-2.51421986332297,
-2.51213975030339,-2.51020081444974,-2.50767353314413,-2.50342783372285,
-2.47122885075476,-2.43578620023354,-2.41829769048525,-2.40946119833998,
-2.40735964264383,-2.40613099296778,-2.40505584991846,-2.40366725197709,
-2.40075442504182,-2.36926629053877,-2.3184592597984,-2.31014901888898,
-2.3040998529636,-2.3014246241393,-2.29946850945367,-2.29766799802435,-2.29476178318676,
-2.28763143438713,-2.23880480649687,-2.19967629084255,-2.19610106332546,
-2.19459175429153,-2.19349936616057,-2.19247321713409,-2.19072970000656,
-2.18599565714715,-2.14618181156768,-2.09848204321019,-2.09208421069137,
-2.08938116470109,-2.08742012077934,-2.08562572765126,-2.08275277023494,
-2.07582227592471,-2.02333086177869,-1.9969984583142,-1.98558223788631,
-1.98330310124768,-1.98204504118789,-1.98097353402213,-1.97962716041026,
-1.9770128019396,-1.96112406487979,-1.95269722264833,-1.91136684888007,
-1.89271083159245,-1.88147841142933,-1.8781274666877,-1.87603123828051,
-1.87409805635767,-1.87160746720959,-1.86748693128449,-1.84054434892272,
-1.79861302725543,-1.78184939889946,-1.77323732522018,-1.77114577576153,
-1.76992890075814,-1.76885161693807,-1.76746704023715,-1.76517806504482,
-1.75150394292382,-1.74978242849758,-1.70241593615213,-1.67144142341111,
-1.66698943453022,-1.66465381635431,-1.6627413266828,-1.66052635305962,
-1.65673879311931,-1.64214417233858,-1.6298786516596,-1.58946761081467,
-1.57061392260565,-1.56131512761951,-1.55917184644827,-1.55794356523527,
-1.55686847296439,-1.5554795820761,-1.55256487524529,-1.52372643522699,
-1.4856166908261,-1.46809095165913,-1.4573497752477,-1.45405209439119,-1.45196768183834,
-1.45003059930798,-1.44751407113299,-1.4433048278966,-1.41283082291991,
-1.36760469595528,-1.35571214220384,-1.35117705443448,-1.34786864607341,
-1.34640616341106,-1.34532146060471,-1.3441325725923,-1.34216662668467,
-1.33576152148236,-1.3342056133521,-1.31961907874268,-1.260577564675,-1.25976204361674),
 .UNSPECIFIED.);
#920=B_SPLINE_CURVE_WITH_KNOTS('',3,(#91735,#91736,#91737,#91738,#91739,
#91740,#91741,#91742),.UNSPECIFIED.,.F.,.F.,(4,2,2,4),(-0.0748537111811377,
-0.0742481347811158,-0.0252918437645686,-0.00062946485106353),
 .UNSPECIFIED.);
#921=B_SPLINE_CURVE_WITH_KNOTS('',3,(#91743,#91744,#91745,#91746,#91747,
#91748,#91749,#91750,#91751,#91752,#91753,#91754,#91755,#91756,#91757,#91758,
#91759,#91760,#91761,#91762,#91763,#91764,#91765,#91766,#91767,#91768,#91769,
#91770,#91771,#91772,#91773,#91774,#91775,#91776,#91777,#91778,#91779,#91780,
#91781,#91782,#91783,#91784,#91785,#91786,#91787,#91788,#91789,#91790,#91791,
#91792,#91793,#91794,#91795,#91796,#91797,#91798,#91799,#91800,#91801,#91802,
#91803,#91804,#91805,#91806,#91807,#91808,#91809,#91810,#91811,#91812,#91813,
#91814,#91815,#91816,#91817,#91818,#91819,#91820,#91821,#91822,#91823,#91824,
#91825,#91826,#91827,#91828,#91829,#91830,#91831,#91832,#91833,#91834,#91835,
#91836,#91837,#91838,#91839,#91840,#91841,#91842,#91843,#91844,#91845,#91846,
#91847,#91848,#91849,#91850,#91851,#91852,#91853,#91854,#91855,#91856,#91857,
#91858,#91859,#91860,#91861,#91862,#91863,#91864,#91865,#91866,#91867,#91868,
#91869,#91870,#91871,#91872,#91873,#91874,#91875,#91876,#91877,#91878,#91879,
#91880,#91881,#91882,#91883,#91884,#91885,#91886,#91887,#91888,#91889,#91890,
#91891,#91892,#91893,#91894,#91895,#91896,#91897,#91898,#91899,#91900,#91901,
#91902,#91903,#91904,#91905,#91906,#91907,#91908,#91909,#91910,#91911,#91912,
#91913,#91914,#91915,#91916,#91917,#91918,#91919,#91920,#91921,#91922,#91923,
#91924,#91925,#91926,#91927,#91928,#91929,#91930,#91931,#91932,#91933,#91934,
#91935,#91936,#91937,#91938,#91939,#91940,#91941,#91942,#91943,#91944,#91945,
#91946,#91947,#91948,#91949,#91950,#91951,#91952,#91953,#91954,#91955,#91956,
#91957,#91958,#91959,#91960,#91961,#91962,#91963,#91964,#91965,#91966,#91967,
#91968,#91969,#91970,#91971,#91972,#91973,#91974,#91975,#91976,#91977,#91978,
#91979,#91980,#91981,#91982,#91983,#91984,#91985,#91986,#91987,#91988,#91989,
#91990,#91991,#91992,#91993,#91994,#91995,#91996,#91997,#91998,#91999,#92000),
 .UNSPECIFIED.,.F.,.F.,(4,2,2,2,2,2,2,2,2,2,2,2,2,2,2,2,2,2,2,2,2,2,2,2,
2,2,2,2,2,2,2,2,2,2,2,2,2,2,2,2,2,2,2,2,2,2,2,2,2,2,2,2,2,2,2,2,2,2,2,2,
2,2,2,2,2,2,2,2,2,2,2,2,2,2,2,2,2,2,2,2,2,2,2,2,2,2,2,2,2,2,2,2,2,2,2,2,
2,2,2,2,2,2,2,2,2,2,2,2,2,2,2,2,2,2,2,2,2,2,2,2,2,2,2,2,2,2,2,2,4),(-2.66791417378201,
-2.66011988777631,-2.65482313930386,-2.65237961614905,-2.65049765042171,
-2.64865683449738,-2.64683032342862,-2.64428978233245,-2.63909831227884,
-2.62658735449175,-2.5749150821746,-2.55607160762977,-2.54677616300546,
-2.54463317126834,-2.54340497810905,-2.54232991213756,-2.54094098819484,
-2.53802597530639,-2.50832788054379,-2.4578760875252,-2.4483865807636,-2.44377906975308,
-2.43999977866059,-2.43782896495123,-2.43781326973063,-2.43779702190874,
-2.43778020143896,-2.43776278742412,-2.43774475824523,-2.43772609151703,
-2.43770676403998,-2.43768675171188,-2.43766602962809,-2.43764457202056,
-2.43762235216574,-2.43759934167047,-2.43757930447203,-2.43755595309751,
-2.43752874547583,-2.43749705356636,-2.43746015098454,-2.43741719944656,
-2.43736298553626,-2.43542216926865,-2.43288003452889,-2.42858165316826,
-2.39345884284186,-2.34449859829081,-2.33479760947715,-2.33262624841412,
-2.3313919405314,-2.33031805948839,-2.32893923323287,-2.32607523268267,
-2.2901166619028,-2.25734989063278,-2.23478976319528,-2.22913613951212,
-2.22656484650643,-2.22462637742261,-2.22279965521206,-2.22025769292186,
-2.21361644443353,-2.15780940066184,-2.1337456447536,-2.12292178675442,
-2.12067774575561,-2.11942747359353,-2.11835548969604,-2.11699940698459,
-2.11485378640741,-2.10381682253215,-2.05259701171859,-2.02388666735185,
-2.01745269554198,-2.01474390319664,-2.01278214780467,-2.01098948279204,
-2.0081244719523,-2.00123993179152,-1.94816229749233,-1.92225391450773,
-1.91094622475129,-1.90867365474704,-1.90741719076193,-1.90634581212781,
-1.90499803307594,-1.90237634137701,-1.88633367703237,-1.88104245191794,
-1.86645752599065,-1.83356411220798,-1.81699649221149,-1.8066836117489,
-1.80343450454297,-1.80136097306187,-1.79942012963745,-1.79687878844678,
-1.79258360740925,-1.75746994548861,-1.70856299624024,-1.69879210687913,
-1.6966157924424,-1.69538031718803,-1.69430647621343,-1.69292908163961,
-1.69007280912309,-1.66727127306139,-1.611660506485,-1.59564836420045,-1.59187872760401,
-1.58969015458288,-1.5877758610531,-1.58540646714517,-1.58177292300582,
-1.56467493167577,-1.55660605266961,-1.52179402174411,-1.49774304356339,
-1.48692288587444,-1.48467916179566,-1.48342900309034,-1.4823570775557,
-1.48100101874928,-1.47834061639203,-1.46128641298507,-1.44267340483334,
-1.40971563401133,-1.40850263276381),.UNSPECIFIED.);
#922=B_SPLINE_CURVE_WITH_KNOTS('',3,(#92002,#92003,#92004,#92005,#92006,
#92007,#92008,#92009,#92010,#92011,#92012,#92013,#92014,#92015,#92016,#92017,
#92018,#92019,#92020,#92021,#92022,#92023,#92024,#92025,#92026,#92027,#92028,
#92029,#92030,#92031,#92032,#92033,#92034,#92035,#92036,#92037,#92038,#92039,
#92040,#92041,#92042,#92043,#92044,#92045,#92046,#92047,#92048,#92049,#92050,
#92051,#92052,#92053,#92054,#92055,#92056,#92057,#92058,#92059,#92060,#92061,
#92062,#92063,#92064,#92065,#92066,#92067,#92068,#92069,#92070,#92071,#92072,
#92073,#92074,#92075,#92076,#92077,#92078,#92079,#92080,#92081,#92082,#92083,
#92084,#92085,#92086,#92087,#92088,#92089,#92090,#92091,#92092,#92093,#92094,
#92095,#92096,#92097,#92098,#92099,#92100,#92101,#92102,#92103,#92104,#92105,
#92106,#92107,#92108,#92109,#92110,#92111,#92112,#92113,#92114,#92115,#92116,
#92117,#92118,#92119,#92120,#92121,#92122,#92123,#92124,#92125,#92126,#92127,
#92128,#92129,#92130,#92131,#92132,#92133,#92134,#92135,#92136,#92137,#92138,
#92139,#92140,#92141,#92142,#92143,#92144,#92145,#92146,#92147,#92148,#92149,
#92150,#92151,#92152,#92153,#92154,#92155,#92156,#92157,#92158,#92159,#92160,
#92161,#92162,#92163,#92164,#92165,#92166,#92167,#92168,#92169,#92170,#92171,
#92172,#92173,#92174,#92175,#92176,#92177,#92178,#92179,#92180,#92181,#92182,
#92183,#92184,#92185,#92186,#92187,#92188,#92189,#92190,#92191,#92192,#92193,
#92194,#92195,#92196,#92197,#92198,#92199,#92200,#92201,#92202,#92203,#92204,
#92205,#92206,#92207,#92208,#92209,#92210,#92211),.UNSPECIFIED.,.F.,.F.,
(4,2,2,2,2,2,2,2,2,2,2,2,2,2,2,2,2,2,2,2,2,2,2,2,2,2,2,2,2,2,2,2,2,2,2,
2,2,2,2,2,2,2,2,2,2,2,2,2,2,2,2,2,2,2,2,2,2,2,2,2,2,2,2,2,2,2,2,2,2,2,2,
2,2,2,2,2,2,2,2,2,2,2,2,2,2,2,2,2,2,2,2,2,2,2,2,2,2,2,2,2,2,2,2,2,4),(-1.25976204361674,
-1.24626789056776,-1.24250620752153,-1.24029737663238,-1.23838472323266,
-1.23604199837598,-1.23155507448113,-1.19919334391832,-1.15901178270338,
-1.15407895720171,-1.13812873676784,-1.13551216621872,-1.1341654469943,
-1.13309408235513,-1.13183667968111,-1.12955997168365,-1.11818207834973,
-1.09199581744802,-1.03926899084753,-1.03235477190914,-1.02948478617842,
-1.02769115130942,-1.02573006110216,-1.02302534229468,-1.01661594655854,
-0.988116698680607,-0.93718442266636,-0.925703276043635,-0.923530854995222,
-0.922166599381747,-0.921093955434373,-0.919849550069128,-0.917632410998708,
-0.907242337329322,-0.884745543786685,-0.826436712066803,-0.820077262709895,
-0.817581121950843,-0.815766391624696,-0.813821068532292,-0.811206787351942,
-0.805316257970909,-0.780974088587364,-0.730305840290646,-0.71407588728807,
-0.711447286952908,-0.710098030610435,-0.709026564900586,-0.707771263015832,
-0.705503988348638,-0.694288065155435,-0.668734702193589,-0.615102399043116,
-0.608259434399044,-0.605401288048424,-0.603609886083817,-0.601647074328424,
-0.598932331757705,-0.592462826313168,-0.538201382963245,-0.502341072333416,
-0.499482572086244,-0.498104806605431,-0.497031003408468,-0.495795949084924,
-0.49362126492952,-0.483872723874646,-0.43492573468846,-0.399782611955477,
-0.395494880052352,-0.392955855919747,-0.391015565965953,-0.388941444641914,
-0.385688942987294,-0.375344324635835,-0.358708038445344,-0.32578784281186,
-0.307703638288777,-0.290152223210228,-0.287474033309213,-0.286114239796449,
-0.285042105394494,-0.283794855511992,-0.281564166852736,-0.270954727217956,
-0.247671400600385,-0.191963501212568,-0.184499084404424,-0.181536679834136,
-0.17972621909234,-0.177896302471686,-0.175389705980593,-0.170057324587429,
-0.162973596288587,-0.145587511867453,-0.0967120992549064,-0.0782146044816004,
-0.0754712688757332,-0.074116472291463,-0.0730447648057392,-0.0717939694947669,
-0.0695468645916382,-0.0586677900867371,-0.0343929976268521,-0.000629544711740993),
 .UNSPECIFIED.);
#923=B_SPLINE_CURVE_WITH_KNOTS('',3,(#92212,#92213,#92214,#92215,#92216,
#92217,#92218,#92219,#92220,#92221,#92222,#92223,#92224,#92225,#92226,#92227,
#92228,#92229,#92230,#92231,#92232,#92233),.UNSPECIFIED.,.F.,.F.,(4,2,2,
2,2,2,2,2,2,2,4),(-2.66775452449513,-2.64242641789711,-2.63929920756027,
-2.6371529728418,-2.63535203504439,-2.63343794716631,-2.63106861207781,
-2.62743479154457,-2.61032817670121,-2.5981367253121,-2.5933285988703),
 .UNSPECIFIED.);
#924=B_SPLINE_CURVE_WITH_KNOTS('',3,(#92238,#92239,#92240,#92241,#92242,
#92243,#92244,#92245,#92246,#92247,#92248,#92249,#92250,#92251,#92252,#92253,
#92254,#92255,#92256,#92257,#92258,#92259,#92260,#92261,#92262,#92263,#92264,
#92265,#92266,#92267,#92268,#92269,#92270,#92271,#92272,#92273,#92274,#92275,
#92276,#92277,#92278,#92279,#92280,#92281,#92282,#92283,#92284,#92285,#92286,
#92287,#92288,#92289,#92290,#92291,#92292,#92293,#92294,#92295,#92296,#92297,
#92298,#92299,#92300,#92301,#92302,#92303,#92304,#92305,#92306,#92307,#92308,
#92309,#92310,#92311,#92312,#92313,#92314,#92315,#92316,#92317,#92318,#92319,
#92320,#92321,#92322,#92323,#92324,#92325,#92326,#92327,#92328,#92329,#92330,
#92331,#92332,#92333,#92334,#92335,#92336,#92337,#92338,#92339,#92340,#92341,
#92342,#92343,#92344,#92345,#92346,#92347,#92348,#92349,#92350,#92351,#92352,
#92353,#92354,#92355,#92356,#92357,#92358,#92359,#92360,#92361,#92362,#92363,
#92364,#92365,#92366,#92367,#92368,#92369,#92370,#92371,#92372,#92373,#92374,
#92375,#92376,#92377,#92378,#92379,#92380,#92381,#92382,#92383,#92384,#92385,
#92386,#92387,#92388,#92389,#92390,#92391,#92392,#92393,#92394,#92395,#92396,
#92397,#92398,#92399,#92400,#92401,#92402,#92403,#92404,#92405,#92406,#92407,
#92408,#92409,#92410,#92411,#92412,#92413,#92414,#92415,#92416,#92417,#92418,
#92419,#92420,#92421,#92422,#92423,#92424,#92425,#92426,#92427,#92428,#92429,
#92430,#92431,#92432,#92433,#92434,#92435,#92436,#92437,#92438,#92439,#92440,
#92441,#92442,#92443,#92444,#92445,#92446,#92447,#92448,#92449,#92450,#92451,
#92452,#92453,#92454,#92455,#92456,#92457,#92458,#92459,#92460,#92461,#92462,
#92463,#92464,#92465,#92466,#92467,#92468,#92469,#92470,#92471),
 .UNSPECIFIED.,.F.,.F.,(4,2,2,2,2,2,2,2,2,2,2,2,2,2,2,2,2,2,2,2,2,2,2,2,
2,2,2,2,2,2,2,2,2,2,2,2,2,2,2,2,2,2,2,2,2,2,2,2,2,2,2,2,2,2,2,2,2,2,2,2,
2,2,2,2,2,2,2,2,2,2,2,2,2,2,2,2,2,2,2,2,2,2,2,2,2,2,2,2,2,2,2,2,2,2,2,2,
2,2,2,2,2,2,2,2,2,2,2,2,2,2,2,2,2,2,2,2,4),(-1.40847047624389,-1.40132353743621,
-1.37516892029172,-1.36379828879407,-1.36152198615809,-1.36026465228302,
-1.35919325578629,-1.35784637524951,-1.35522913707094,-1.33926698399098,
-1.33432293362518,-1.32867696470249,-1.28171646060601,-1.28027359363999,
-1.26123211568003,-1.25747075147992,-1.25506192387486,-1.2531441471841,
-1.25098196098015,-1.24733225562943,-1.23288148699016,-1.18249250495218,
-1.15282399940257,-1.14990948108709,-1.14852070342273,-1.14744570571998,
-1.14621754955971,-1.14407451199863,-1.13477746815999,-1.11592581565445,
-1.07547220613324,-1.06319340351377,-1.04861348388434,-1.04482747636013,
-1.04261300281901,-1.04070069725353,-1.03836499232274,-1.03391187464162,
-1.00287553876273,-0.954897375402384,-0.940308395336562,-0.937976024716122,
-0.93657877735863,-0.935499972890641,-0.934290700817501,-0.932232964378333,
-0.924037414039032,-0.908470911388692,-0.866886481247444,-0.837982824145689,
-0.833811354540374,-0.831306003015753,-0.829370803329042,-0.827281765548493,
-0.823962525089069,-0.813022721552837,-0.795045740404755,-0.744623372304772,
-0.728417185128947,-0.725789296870255,-0.724440098321774,-0.723368517189738,
-0.722112893355214,-0.719844564322076,-0.708613860326878,-0.683005317714944,
-0.629442127697143,-0.622592155377476,-0.6197326437578,-0.617940839776557,
-0.615977953404556,-0.613263780767158,-0.606798844079358,-0.552721149169341,
-0.516660503930821,-0.51380070335242,-0.512422583726572,-0.511348632467156,
-0.510113552226802,-0.507939167386879,-0.498197653159695,-0.449237789918328,
-0.414102810569857,-0.409806355515815,-0.407264645382177,-0.405323730871823,
-0.403250326791116,-0.40000184254462,-0.389694422842742,-0.37314119418427,
-0.340287527160839,-0.327286384381564,-0.304664081988268,-0.301812395071588,
-0.300435955411729,-0.299362264349971,-0.298126298268855,-0.295947517236464,
-0.286139319552388,-0.237241787200406,-0.202131568657589,-0.197834505157912,
-0.195292756386959,-0.193351997355742,-0.191344263310538,-0.188242470562931,
-0.18461585200755,-0.1778196522977,-0.161438230576098,-0.128729478564262,
-0.0927003701199963,-0.0898402860636551,-0.0884622742363991,-0.0873885216651818,
-0.0861537993203325,-0.0839803536168609,-0.0748537111811377),
 .UNSPECIFIED.);
#925=B_SPLINE_CURVE_WITH_KNOTS('',3,(#92472,#92473,#92474,#92475,#92476,
#92477,#92478,#92479,#92480,#92481,#92482,#92483,#92484,#92485,#92486,#92487,
#92488,#92489,#92490,#92491,#92492,#92493,#92494,#92495,#92496,#92497,#92498,
#92499,#92500,#92501,#92502,#92503,#92504,#92505,#92506,#92507,#92508,#92509,
#92510,#92511,#92512,#92513,#92514,#92515,#92516,#92517,#92518,#92519,#92520,
#92521,#92522,#92523,#92524,#92525,#92526,#92527,#92528,#92529,#92530,#92531,
#92532,#92533,#92534,#92535,#92536,#92537,#92538,#92539,#92540,#92541,#92542,
#92543,#92544,#92545,#92546,#92547,#92548,#92549,#92550,#92551,#92552,#92553,
#92554,#92555,#92556,#92557,#92558,#92559,#92560,#92561,#92562,#92563,#92564,
#92565,#92566,#92567,#92568,#92569,#92570,#92571,#92572,#92573,#92574,#92575,
#92576,#92577,#92578,#92579,#92580,#92581,#92582,#92583,#92584,#92585,#92586,
#92587,#92588,#92589,#92590,#92591,#92592,#92593,#92594,#92595,#92596,#92597,
#92598,#92599,#92600,#92601,#92602,#92603,#92604,#92605,#92606,#92607,#92608,
#92609,#92610,#92611,#92612,#92613,#92614,#92615,#92616,#92617,#92618,#92619,
#92620,#92621,#92622,#92623,#92624,#92625,#92626,#92627,#92628,#92629,#92630,
#92631,#92632,#92633,#92634,#92635,#92636,#92637,#92638,#92639,#92640,#92641,
#92642,#92643,#92644,#92645,#92646,#92647,#92648,#92649,#92650,#92651,#92652,
#92653,#92654,#92655,#92656,#92657,#92658,#92659,#92660,#92661,#92662,#92663,
#92664,#92665,#92666,#92667,#92668,#92669,#92670,#92671,#92672,#92673,#92674,
#92675,#92676,#92677,#92678,#92679,#92680,#92681,#92682,#92683,#92684,#92685,
#92686,#92687,#92688,#92689,#92690,#92691,#92692,#92693,#92694,#92695,#92696,
#92697,#92698,#92699),.UNSPECIFIED.,.F.,.F.,(4,2,2,2,2,2,2,2,2,2,2,2,2,
2,2,2,2,2,2,2,2,2,2,2,2,2,2,2,2,2,2,2,2,2,2,2,2,2,2,2,2,2,2,2,2,2,2,2,2,
2,2,2,2,2,2,2,2,2,2,2,2,2,2,2,2,2,2,2,2,2,2,2,2,2,2,2,2,2,2,2,2,2,2,2,2,
2,2,2,2,2,2,2,2,2,2,2,2,2,2,2,2,2,2,2,2,2,2,2,2,2,2,2,2,4),(-2.5933285988703,
-2.5713850135869,-2.53465311063345,-2.53109031662975,-2.52958349833753,
-2.52849187727579,-2.52746562274084,-2.52572015644279,-2.52097054031788,
-2.48223390396735,-2.45387433170764,-2.43819312672754,-2.43160235540862,
-2.42655929218752,-2.42411494514773,-2.42218777269432,-2.42033606711082,
-2.41715941167392,-2.40829252768649,-2.40629415126029,-2.34856880498957,
-2.32972682356652,-2.32043266344886,-2.31829012472644,-2.317062216487,-2.31598741641377,
-2.31459885778916,-2.31168468857804,-2.28166275286212,-2.23038397264264,
-2.22154907325308,-2.21514345516761,-2.21243963202807,-2.21047893936624,
-2.20868549839706,-2.20581544124244,-2.19889905323656,-2.14626659808653,
-2.12005397553798,-2.10866956701911,-2.10639278493715,-2.10513549074595,
-2.10406431256044,-2.10271794113495,-2.1001023809276,-2.08416605388714,
-2.07847457312878,-2.06416907003625,-2.0312824157178,-2.01472038767583,
-2.00441034798618,-2.00116179537938,-1.99908853605496,-1.99714788992904,
-1.99460672420656,-1.99031165400152,-1.95517416366392,-1.90618645682308,
-1.8965182238893,-1.89434913551788,-1.89311533307694,-1.89204138658685,
-1.89066181467709,-1.88843860206047,-1.87604928123388,-1.8729879344285,
-1.87278968000235,-1.86592217170183,-1.85218958767901,-1.81930667198492,
-1.80275079500559,-1.79244333503107,-1.78919493039683,-1.78712160572002,
-1.78518078616931,-1.78263923138216,-1.77834314051044,-1.74314810052261,
-1.69397665233024,-1.68451701778498,-1.68236243356225,-1.68113177021427,
-1.68005725122178,-1.67867259929824,-1.67577906732336,-1.64974430551735,
-1.61157686690087,-1.58254861834206,-1.57815295809465,-1.57582935992611,
-1.57391773255557,-1.57169358403674,-1.56786528472473,-1.55280376810564,
-1.50063474161939,-1.48178895401521,-1.47249301199153,-1.47035008983546,
-1.46912196625316,-1.46804698056332,-1.4666581859312,-1.46374353480768,
-1.43369701143151,-1.38235474301257,-1.36901439214692,-1.36545930408266,
-1.36331812272215,-1.36139681622109,-1.35895345466862,-1.35507885020997,
-1.33400441802887,-1.27618777129635,-1.26122677147129,-1.25979232650984),
 .UNSPECIFIED.);
#926=B_SPLINE_CURVE_WITH_KNOTS('',3,(#92705,#92706,#92707,#92708),
 .UNSPECIFIED.,.F.,.F.,(4,4),(120.339865594546,120.689851222923),
 .UNSPECIFIED.);
#927=B_SPLINE_CURVE_WITH_KNOTS('',3,(#92709,#92710,#92711,#92712,#92713,
#92714,#92715,#92716,#92717,#92718,#92719,#92720,#92721,#92722,#92723,#92724,
#92725,#92726,#92727,#92728,#92729,#92730,#92731,#92732,#92733,#92734,#92735,
#92736,#92737,#92738,#92739,#92740,#92741,#92742,#92743,#92744,#92745,#92746,
#92747,#92748,#92749,#92750,#92751,#92752,#92753,#92754,#92755,#92756,#92757,
#92758,#92759,#92760,#92761,#92762,#92763,#92764,#92765,#92766,#92767,#92768,
#92769,#92770,#92771,#92772,#92773,#92774,#92775,#92776,#92777,#92778,#92779,
#92780,#92781,#92782,#92783,#92784,#92785,#92786,#92787,#92788,#92789,#92790,
#92791,#92792,#92793,#92794,#92795,#92796,#92797,#92798,#92799,#92800,#92801,
#92802,#92803,#92804,#92805,#92806,#92807,#92808,#92809,#92810,#92811,#92812,
#92813,#92814,#92815,#92816,#92817,#92818,#92819,#92820,#92821,#92822,#92823,
#92824,#92825,#92826,#92827,#92828,#92829,#92830,#92831,#92832,#92833,#92834,
#92835,#92836,#92837,#92838,#92839,#92840,#92841,#92842,#92843,#92844,#92845,
#92846,#92847,#92848,#92849,#92850,#92851,#92852,#92853,#92854,#92855,#92856,
#92857,#92858,#92859,#92860,#92861,#92862,#92863,#92864,#92865,#92866,#92867,
#92868,#92869,#92870,#92871,#92872,#92873,#92874,#92875,#92876,#92877,#92878,
#92879,#92880,#92881,#92882,#92883,#92884,#92885,#92886,#92887,#92888,#92889,
#92890,#92891,#92892,#92893,#92894,#92895,#92896,#92897,#92898,#92899,#92900,
#92901,#92902,#92903,#92904,#92905,#92906,#92907,#92908,#92909,#92910,#92911,
#92912,#92913,#92914,#92915,#92916,#92917,#92918,#92919,#92920,#92921,#92922,
#92923,#92924,#92925,#92926),.UNSPECIFIED.,.F.,.F.,(4,2,2,2,2,2,2,2,2,2,
2,2,2,2,2,2,2,2,2,2,2,2,2,2,2,2,2,2,2,2,2,2,2,2,2,2,2,2,2,2,2,2,2,2,2,2,
2,2,2,2,2,2,2,2,2,2,2,2,2,2,2,2,2,2,2,2,2,2,2,2,2,2,2,2,2,2,2,2,2,2,2,2,
2,2,2,2,2,2,2,2,2,2,2,2,2,2,2,2,2,2,2,2,2,2,2,2,2,2,4),(-2.6676132306845,
-2.64338324964044,-2.63625129884618,-2.63446038505705,-2.63324541682247,
-2.63223633571066,-2.6311617534206,-2.62977571315959,-2.6268746985405,-2.59995420508059,
-2.58627103785683,-2.57475029045549,-2.54617396108281,-2.53227586374139,
-2.52867234232268,-2.52652047555009,-2.52460120080779,-2.52217616405178,
-2.51744440404228,-2.48000654891398,-2.4296553031146,-2.42318139015113,
-2.42128996035042,-2.42027899069394,-2.4192057173042,-2.4178340292279,-2.41563706192836,
-2.40380017738245,-2.34640349851753,-2.32983966017304,-2.31952880759204,
-2.31628016582027,-2.31420688969781,-2.31226625601916,-2.30972514723753,
-2.30543026435078,-2.27030646223537,-2.2213615195394,-2.21164313595713,
-2.2094705913563,-2.2082360302315,-2.20716219796055,-2.20578378645264,-2.20292186238522,
-2.16686121967266,-2.13412928611118,-2.11162313130751,-2.10597684092514,
-2.10340691167659,-2.10146866777271,-2.09964156741848,-2.09709813098796,
-2.09044736649844,-2.03473181990158,-2.01060894251548,-1.99976919264833,
-1.99752420514233,-1.99627373433666,-1.99520178269729,-1.99384600061808,
-1.99118706889081,-1.9741750205537,-1.92396840007978,-1.90638766610325,
-1.89562291339788,-1.89232308685835,-1.89023849623266,-1.88830206139456,
-1.88578752850923,-1.88158416064999,-1.85133516455136,-1.79985544975948,
-1.78786931914926,-1.78555913142079,-1.78429451629283,-1.7832237543346,
-1.7818863064808,-1.77980150186393,-1.76970633312755,-1.76421748453725,
-1.75679098752139,-1.74328323594381,-1.71040120074048,-1.69384735844554,
-1.68354069909977,-1.68029229857287,-1.67821891684895,-1.67627800197455,
-1.67373626185901,-1.66943972208803,-1.63422231967192,-1.58497686288309,
-1.57559917072624,-1.57345036347776,-1.57222094128947,-1.57114616868146,
-1.56975942826541,-1.56751268574364,-1.55467956023738,-1.55251362126544,
-1.50523274194232,-1.47670830799613,-1.47029627829055,-1.46759106545853,
-1.46562984425439,-1.46383624997819,-1.46096666712225,-1.45405514491847,
-1.40847047624389),.UNSPECIFIED.);
#928=B_SPLINE_CURVE_WITH_KNOTS('',3,(#92928,#92929,#92930,#92931,#92932,
#92933,#92934,#92935,#92936,#92937,#92938,#92939,#92940,#92941,#92942,#92943,
#92944,#92945,#92946,#92947,#92948,#92949,#92950,#92951,#92952,#92953,#92954,
#92955,#92956,#92957,#92958,#92959,#92960,#92961,#92962,#92963,#92964,#92965,
#92966,#92967,#92968,#92969,#92970,#92971,#92972,#92973,#92974,#92975,#92976,
#92977,#92978,#92979,#92980,#92981,#92982,#92983,#92984,#92985,#92986,#92987,
#92988,#92989,#92990,#92991,#92992,#92993,#92994,#92995,#92996,#92997,#92998,
#92999,#93000,#93001,#93002,#93003,#93004,#93005,#93006,#93007,#93008,#93009,
#93010,#93011,#93012,#93013,#93014,#93015,#93016,#93017,#93018,#93019,#93020,
#93021,#93022,#93023,#93024,#93025,#93026,#93027,#93028,#93029,#93030,#93031,
#93032,#93033,#93034,#93035,#93036,#93037,#93038,#93039,#93040,#93041,#93042,
#93043,#93044,#93045,#93046,#93047,#93048,#93049,#93050,#93051,#93052,#93053,
#93054,#93055,#93056,#93057,#93058,#93059,#93060,#93061,#93062,#93063,#93064,
#93065,#93066,#93067,#93068,#93069,#93070,#93071,#93072,#93073,#93074,#93075,
#93076,#93077,#93078,#93079,#93080,#93081,#93082,#93083,#93084,#93085,#93086,
#93087,#93088,#93089,#93090,#93091,#93092,#93093,#93094,#93095,#93096,#93097,
#93098,#93099,#93100,#93101,#93102,#93103,#93104,#93105,#93106,#93107,#93108,
#93109,#93110,#93111,#93112,#93113,#93114,#93115,#93116,#93117,#93118,#93119,
#93120,#93121,#93122,#93123,#93124,#93125,#93126,#93127,#93128,#93129,#93130,
#93131,#93132,#93133,#93134,#93135,#93136,#93137,#93138,#93139,#93140,#93141,
#93142,#93143,#93144,#93145,#93146,#93147,#93148,#93149),.UNSPECIFIED.,
 .F.,.F.,(4,2,2,2,2,2,2,2,2,2,2,2,2,2,2,2,2,2,2,2,2,2,2,2,2,2,2,2,2,2,2,
2,2,2,2,2,2,2,2,2,2,2,2,2,2,2,2,2,2,2,2,2,2,2,2,2,2,2,2,2,2,2,2,2,2,2,2,
2,2,2,2,2,2,2,2,2,2,2,2,2,2,2,2,2,2,2,2,2,2,2,2,2,2,2,2,2,2,2,2,2,2,2,2,
2,2,2,2,2,2,2,4),(-1.25979232650984,-1.25887869460015,-1.257476860145,-1.25639744792124,
-1.25519075593238,-1.25314458020512,-1.24508694146706,-1.22990728012695,
-1.19000982666574,-1.15896499636262,-1.15474332494294,-1.15222331171263,
-1.15028583896795,-1.14820325862736,-1.14491325930357,-1.13423929197516,
-1.11686740825185,-1.06816235716437,-1.06164763258783,-1.0490240788199,
-1.04678825533364,-1.04540478332008,-1.04433032453203,-1.04309877832677,
-1.04094038551765,-1.03142842291219,-0.982273251324694,-0.947076531422124,
-0.942780070160903,-0.940238384086857,-0.93829750391988,-0.936224152011337,
-0.932975781834942,-0.922668996577683,-0.906117046141392,-0.873264817914013,
-0.860348802374789,-0.837642971990654,-0.834789282164727,-0.83341246536707,
-0.832338757489996,-0.83110308537762,-0.828925572918464,-0.819135550155312,
-0.770223866655688,-0.735105735444874,-0.730810710321477,-0.728269578319782,
-0.726328951071264,-0.724255704345183,-0.721007154466157,-0.710696895442398,
-0.694136605118975,-0.661279490593475,-0.64750719754613,-0.640733949821207,
-0.638831069639443,-0.62518506433143,-0.622898065909665,-0.62151431800853,
-0.620437452947476,-0.619220807393344,-0.617129085688284,-0.608508670809888,
-0.59171518152647,-0.549743130652129,-0.522869190623174,-0.518751294507463,
-0.516261958164872,-0.514329534457623,-0.512233912916489,-0.50888346897489,
-0.497648193390317,-0.478985423521949,-0.438419364079774,-0.413804379442228,
-0.410920235105802,-0.409537569025515,-0.40846342264519,-0.407231882225821,
-0.405072666057842,-0.395543776896042,-0.346417434759987,-0.311234436668114,
-0.306939103201581,-0.304398064758778,-0.302457667881574,-0.300384821339433,
-0.297137220157524,-0.286832682948307,-0.270284160281976,-0.237937392265993,
-0.201815491921998,-0.198960466844357,-0.197583579605201,-0.196557065839457,
-0.195363678496637,-0.193380718674547,-0.190940950290321,-0.185982530594728,
-0.172431551898505,-0.149608300831557,-0.103071676025014,-0.0958752177108702,
-0.0929587265886628,-0.0911569205292869,-0.0892033973504025,-0.0865388835416779,
-0.0803615103261198,-0.0537591566479666,-0.00062960350502436),
 .UNSPECIFIED.);
#929=B_SPLINE_CURVE_WITH_KNOTS('',3,(#93150,#93151,#93152,#93153,#93154,
#93155,#93156,#93157,#93158,#93159,#93160,#93161,#93162,#93163,#93164,#93165,
#93166,#93167,#93168,#93169,#93170,#93171,#93172,#93173),.UNSPECIFIED.,
 .F.,.F.,(4,2,2,2,2,2,2,2,2,2,2,4),(-2.66811719344424,-2.66005991212222,
-2.65570245956423,-2.65428938514948,-2.65322207097606,-2.65219180145323,
-2.65101182025699,-2.64908649323056,-2.64302060358045,-2.64173852058932,
-2.63393766869622,-2.59385608721132),.UNSPECIFIED.);
#930=B_SPLINE_CURVE_WITH_KNOTS('',3,(#93179,#93180,#93181,#93182,#93183,
#93184,#93185,#93186,#93187,#93188,#93189,#93190,#93191),.UNSPECIFIED.,
 .F.,.F.,(4,3,3,3,4),(114.057240355212,114.163813746624,114.270250447226,
114.376547360035,114.406671945289),.UNSPECIFIED.);
#931=B_SPLINE_CURVE_WITH_KNOTS('',3,(#93192,#93193,#93194,#93195,#93196,
#93197,#93198,#93199,#93200,#93201),.UNSPECIFIED.,.F.,.F.,(4,1,1,1,1,1,
1,4),(114.406674973133,114.866191745616,115.865028195577,116.863864645539,
117.862701095501,118.861537545463,119.860373995425,120.339865594546),
 .UNSPECIFIED.);
#932=B_SPLINE_CURVE_WITH_KNOTS('',3,(#93202,#93203,#93204,#93205,#93206,
#93207,#93208,#93209,#93210,#93211,#93212,#93213,#93214,#93215,#93216,#93217,
#93218,#93219,#93220,#93221,#93222,#93223,#93224,#93225,#93226,#93227,#93228,
#93229,#93230,#93231,#93232,#93233,#93234,#93235,#93236,#93237,#93238,#93239,
#93240,#93241,#93242,#93243,#93244,#93245,#93246,#93247,#93248,#93249,#93250,
#93251,#93252,#93253,#93254,#93255,#93256,#93257,#93258,#93259,#93260,#93261,
#93262,#93263,#93264,#93265,#93266,#93267,#93268,#93269,#93270,#93271,#93272,
#93273,#93274,#93275,#93276,#93277,#93278,#93279,#93280,#93281,#93282,#93283,
#93284,#93285,#93286,#93287,#93288,#93289,#93290,#93291,#93292,#93293,#93294,
#93295,#93296,#93297,#93298,#93299,#93300,#93301,#93302,#93303,#93304,#93305,
#93306,#93307,#93308,#93309,#93310,#93311,#93312,#93313,#93314,#93315,#93316,
#93317,#93318,#93319,#93320,#93321,#93322,#93323,#93324,#93325,#93326,#93327,
#93328,#93329,#93330,#93331,#93332,#93333,#93334,#93335,#93336,#93337,#93338,
#93339,#93340,#93341,#93342,#93343,#93344,#93345,#93346,#93347,#93348,#93349,
#93350,#93351,#93352,#93353,#93354,#93355,#93356,#93357,#93358,#93359,#93360,
#93361,#93362,#93363,#93364,#93365,#93366,#93367,#93368,#93369,#93370,#93371,
#93372,#93373,#93374,#93375,#93376,#93377,#93378,#93379,#93380,#93381,#93382,
#93383,#93384,#93385,#93386,#93387,#93388,#93389,#93390,#93391,#93392,#93393,
#93394,#93395,#93396,#93397,#93398,#93399,#93400,#93401,#93402,#93403,#93404,
#93405,#93406,#93407,#93408,#93409,#93410,#93411,#93412,#93413,#93414,#93415,
#93416,#93417,#93418,#93419,#93420,#93421,#93422,#93423,#93424,#93425,#93426,
#93427,#93428,#93429,#93430,#93431,#93432,#93433,#93434,#93435,#93436,#93437,
#93438,#93439,#93440,#93441,#93442,#93443,#93444,#93445,#93446,#93447,#93448,
#93449,#93450,#93451,#93452,#93453,#93454,#93455,#93456,#93457,#93458,#93459,
#93460,#93461,#93462,#93463,#93464,#93465),.UNSPECIFIED.,.F.,.F.,(4,2,2,
2,2,2,2,2,2,2,2,2,2,2,2,2,2,2,2,2,2,2,2,2,2,2,2,2,2,2,2,2,2,2,2,2,2,2,2,
2,2,2,2,2,2,2,2,2,2,2,2,2,2,2,2,2,2,2,2,2,2,2,2,2,2,2,2,2,2,2,2,2,2,2,2,
2,2,2,2,2,2,2,2,2,2,2,2,2,2,2,2,2,2,2,2,2,2,2,2,2,2,2,2,2,2,2,2,2,2,2,2,
2,2,2,2,2,2,2,2,2,2,2,2,2,2,2,2,2,2,2,2,4),(-2.59385608721132,-2.58073141970544,
-2.56298814981683,-2.55215092037623,-2.54884238281251,-2.54675539781623,
-2.54481887954915,-2.5423072697976,-2.53811544119408,-2.50862542056458,
-2.46750352282329,-2.45206722689791,-2.44665242939645,-2.44405337358974,
-2.44194651736327,-2.44073373600743,-2.44073062156546,-2.44072748826993,
-2.44072433601563,-2.44072116450774,-2.44071797359581,-2.44071476316554,
-2.44071153318834,-2.44070828334381,-2.44070501359305,-2.44070172383806,
-2.44069841395613,-2.44069508393363,-2.44069174629681,-2.4406883941216,
-2.44068502069543,-2.4406816144313,-2.43965466462533,-2.43827707804931,
-2.43541983131054,-2.39931639114125,-2.36659149996972,-2.34409952785361,
-2.33845486533222,-2.33588506236258,-2.33394666324203,-2.33211923237434,
-2.32957503997356,-2.32292052484272,-2.2672286582859,-2.24308328186017,
-2.23223698312491,-2.22999141970881,-2.22874073730073,-2.22766867154095,
-2.22631283141247,-2.22416824302766,-2.21315034930059,-2.1618752647196,
-2.13318530443709,-2.1267534515289,-2.12404485052406,-2.12208297939977,
-2.12029003371052,-2.11742419385461,-2.11053569053077,-2.05749493328063,
-2.031554467432,-2.0202381164397,-2.01796488263818,-2.01670819640877,-2.01563671615603,
-2.01428892117752,-2.01166752769492,-1.99563230439476,-1.99028317553407,
-1.97574260730953,-1.94284634505356,-1.9262776566299,-1.91596400417879,
-1.91271459697753,-1.91064086041,-1.90869981544901,-1.90615819655644,-1.90186251522844,
-1.86674067372041,-1.81781469934133,-1.8080594027981,-1.80588400101227,
-1.80464864891295,-1.80357466208422,-1.80219674977035,-1.79933826555392,
-1.76340771202465,-1.73061857273192,-1.70802945119765,-1.70237137031944,
-1.69979894310503,-1.69785998213037,-1.6960330631888,-1.69349125523593,
-1.68685295790775,-1.63098734605901,-1.59816027156498,-1.59461368759316,
-1.59310930107685,-1.59201777316917,-1.59099027313349,-1.5892398223757,
-1.5844601020464,-1.54728119547981,-1.4970121043773,-1.49060955745954,-1.48790574339682,
-1.48594458825318,-1.48415040087986,-1.48127844389249,-1.47435382986105,
-1.42178270642939,-1.39550755450345,-1.38410585480144,-1.38182757439701,
-1.38056971438782,-1.37949821256404,-1.37815163580577,-1.37553626755946,
-1.35961501635281,-1.35511257552246,-1.33454869744324,-1.28619252276872,
-1.27904322479569,-1.27613386515458,-1.27433279439379,-1.27237717430474,
-1.26970459846511,-1.26348490559208,-1.26001673248898),.UNSPECIFIED.);
#933=B_SPLINE_CURVE_WITH_KNOTS('',3,(#93471,#93472,#93473,#93474,#93475,
#93476,#93477,#93478,#93479,#93480,#93481,#93482,#93483,#93484,#93485,#93486,
#93487,#93488,#93489,#93490),.UNSPECIFIED.,.F.,.F.,(4,2,2,2,2,2,2,2,2,4),
(-0.0747504804368338,-0.0610229392307608,-0.0562870041952136,-0.0545435807646292,
-0.0535177048167566,-0.0524257920513701,-0.0509174388803607,-0.049229620013134,
-0.0462824091130108,-0.000629118632090094),.UNSPECIFIED.);
#934=B_SPLINE_CURVE_WITH_KNOTS('',3,(#93491,#93492,#93493,#93494,#93495,
#93496,#93497,#93498,#93499,#93500,#93501,#93502,#93503,#93504,#93505,#93506,
#93507,#93508,#93509,#93510,#93511,#93512,#93513,#93514,#93515,#93516,#93517,
#93518,#93519,#93520,#93521,#93522,#93523,#93524,#93525,#93526,#93527,#93528,
#93529,#93530,#93531,#93532,#93533,#93534,#93535,#93536,#93537,#93538,#93539,
#93540,#93541,#93542,#93543,#93544,#93545,#93546,#93547,#93548,#93549,#93550,
#93551,#93552,#93553,#93554,#93555,#93556,#93557,#93558,#93559,#93560,#93561,
#93562,#93563,#93564,#93565,#93566,#93567,#93568,#93569,#93570,#93571,#93572,
#93573,#93574,#93575,#93576,#93577,#93578,#93579,#93580,#93581,#93582,#93583,
#93584,#93585,#93586,#93587,#93588,#93589,#93590,#93591,#93592,#93593,#93594,
#93595,#93596,#93597,#93598,#93599,#93600,#93601,#93602,#93603,#93604,#93605,
#93606,#93607,#93608,#93609,#93610,#93611,#93612,#93613,#93614,#93615,#93616,
#93617,#93618,#93619,#93620,#93621,#93622,#93623,#93624,#93625,#93626,#93627,
#93628,#93629,#93630,#93631,#93632,#93633,#93634,#93635,#93636,#93637,#93638,
#93639,#93640,#93641,#93642,#93643,#93644,#93645,#93646,#93647,#93648,#93649,
#93650,#93651,#93652,#93653,#93654,#93655,#93656,#93657,#93658,#93659,#93660,
#93661,#93662,#93663,#93664,#93665,#93666,#93667,#93668,#93669,#93670,#93671),
 .UNSPECIFIED.,.F.,.F.,(4,3,3,3,3,3,3,3,3,3,3,3,3,3,3,3,3,3,3,3,3,3,3,3,
3,3,3,3,3,3,3,3,3,3,3,3,3,3,3,3,3,3,3,3,3,3,3,3,3,3,3,3,3,3,3,3,3,3,3,3,
4),(108.12348663811,108.225421296431,108.327291076164,108.429131491865,
108.530978014042,108.632930880402,108.734945943835,108.837130903884,108.873173045844,
108.976567782892,109.079809065007,109.1829290304,109.285983598609,109.389006806967,
109.492032649639,109.595165416418,109.698354507828,109.80172650121,109.872009495806,
109.975404232854,110.078645514969,110.181765480362,110.284820048571,110.387843256928,
110.490869099601,110.594001866379,110.697190957789,110.800562951171,110.870845945768,
110.974240682816,111.077481964931,111.180601930323,111.283656498532,111.38667970689,
111.489705549562,111.59283831634,111.69602740775,111.799399401132,111.86968239573,
111.973077132778,112.076318414893,112.179438380285,112.282492948494,112.385516156852,
112.488541999524,112.591674766302,112.694863857712,112.798235851094,112.868518845692,
112.97191358274,113.075154864855,113.178274830247,113.281329398456,113.384352606814,
113.487378449486,113.590511216265,113.693700307674,113.797072301056,113.867355295654,
113.974272639427,114.057240355212),.UNSPECIFIED.);
#935=B_SPLINE_CURVE_WITH_KNOTS('',3,(#93673,#93674,#93675,#93676,#93677,
#93678,#93679,#93680,#93681,#93682,#93683,#93684,#93685,#93686,#93687,#93688,
#93689,#93690,#93691,#93692,#93693,#93694,#93695,#93696,#93697,#93698,#93699,
#93700,#93701,#93702,#93703,#93704,#93705,#93706,#93707,#93708,#93709,#93710,
#93711,#93712,#93713,#93714,#93715,#93716,#93717,#93718,#93719,#93720,#93721,
#93722,#93723,#93724,#93725,#93726,#93727,#93728,#93729,#93730,#93731,#93732,
#93733,#93734,#93735,#93736,#93737,#93738,#93739,#93740,#93741,#93742,#93743,
#93744,#93745,#93746,#93747,#93748,#93749,#93750,#93751,#93752,#93753,#93754,
#93755,#93756,#93757,#93758,#93759,#93760,#93761,#93762,#93763,#93764,#93765,
#93766,#93767,#93768,#93769,#93770,#93771,#93772,#93773,#93774,#93775,#93776,
#93777,#93778,#93779,#93780,#93781,#93782,#93783,#93784,#93785,#93786,#93787,
#93788,#93789,#93790,#93791,#93792,#93793,#93794,#93795,#93796,#93797,#93798,
#93799,#93800,#93801,#93802,#93803,#93804,#93805,#93806,#93807,#93808,#93809,
#93810,#93811,#93812,#93813,#93814,#93815,#93816,#93817,#93818,#93819,#93820,
#93821,#93822,#93823,#93824,#93825,#93826,#93827,#93828,#93829,#93830,#93831,
#93832,#93833,#93834,#93835,#93836,#93837,#93838,#93839,#93840,#93841,#93842,
#93843,#93844,#93845,#93846,#93847,#93848,#93849,#93850,#93851,#93852,#93853,
#93854,#93855,#93856,#93857,#93858,#93859,#93860,#93861,#93862,#93863,#93864,
#93865,#93866,#93867,#93868,#93869,#93870,#93871,#93872,#93873,#93874,#93875,
#93876,#93877,#93878,#93879,#93880,#93881,#93882,#93883,#93884),
 .UNSPECIFIED.,.F.,.F.,(4,2,2,2,2,2,2,2,2,2,2,2,2,2,2,2,2,2,2,2,2,2,2,2,
2,2,2,2,2,2,2,2,2,2,2,2,2,2,2,2,2,2,2,2,2,2,2,2,2,2,2,2,2,2,2,2,2,2,2,2,
2,2,2,2,2,2,2,2,2,2,2,2,2,2,2,2,2,2,2,2,2,2,2,2,2,2,2,2,2,2,2,2,2,2,2,2,
2,2,2,2,2,2,2,2,2,4),(-1.26001673248898,-1.23655150319919,-1.1960244005873,
-1.17303176546317,-1.17017627503209,-1.16879893880593,-1.16772499008992,
-1.16648922628762,-1.1643119961818,-1.15453060214934,-1.10560003838702,
-1.0704718400195,-1.06617590381112,-1.06363424451392,-1.0616932213409,-1.05961955819117,
-1.05637036951425,-1.04605819850218,-1.02949494693346,-0.996631493386167,
-0.982888777196495,-0.97603751757564,-0.975722598573606,-0.970126884729276,
-0.960136099439734,-0.958058402905608,-0.956723082636457,-0.955652354111854,
-0.95438582607862,-0.952067046950757,-0.93992193780193,-0.886829788270533,
-0.858243183207196,-0.854080297338155,-0.851577575854991,-0.849642918693378,
-0.847552988978721,-0.844229155057207,-0.833245225473433,-0.815166213195005,
-0.765171947559398,-0.748719770289822,-0.746082303757109,-0.744731118606094,
-0.743659491677619,-0.742405584500435,-0.740144827460915,-0.729041271701423,
-0.703921333791985,-0.649652501817749,-0.642863142352808,-0.640013817473809,
-0.63822396949094,-0.636259643748768,-0.633536870067639,-0.627019737160957,
-0.597610422704946,-0.547778395772928,-0.536270427898126,-0.534096518244313,
-0.532731845752754,-0.53165921532109,-0.530415215220287,-0.528199753886121,
-0.517834773527705,-0.495425778723237,-0.436976136933484,-0.430637133734412,
-0.428144493578436,-0.426330729075971,-0.424384955839965,-0.421767476504563,
-0.415858630299923,-0.391374517538276,-0.340791600172706,-0.324645044531388,
-0.322019897969256,-0.320671425051768,-0.319600062427207,-0.31834428032371,
-0.316074615292846,-0.304815993342912,-0.279095691977376,-0.225710228401517,
-0.218851161607306,-0.216045421859833,-0.214085270360473,-0.212146077489487,
-0.210185605847257,-0.20510920916554,-0.163994077671629,-0.115019541214979,
-0.110791312769733,-0.109127212088262,-0.10811666717333,-0.107013195298084,
-0.105442007963851,-0.101489753644222,-0.0819012664742417,-0.0267278938264957,
-0.0187639942637725,-0.00802108705316168,-0.00466632877897281,-0.00258130086811506,
-0.00128118378586622,-0.000628942594787886),.UNSPECIFIED.);
#936=B_SPLINE_CURVE_WITH_KNOTS('',3,(#93885,#93886,#93887,#93888,#93889,
#93890,#93891,#93892,#93893,#93894,#93895,#93896,#93897),.UNSPECIFIED.,
 .F.,.F.,(4,3,3,3,4),(-104.372003947921,-104.263735348689,-104.155311094115,
-104.04663122551,-104.022525394709),.UNSPECIFIED.);
#937=B_SPLINE_CURVE_WITH_KNOTS('',3,(#93902,#93903,#93904,#93905,#93906,
#93907,#93908,#93909,#93910,#93911,#93912,#93913,#93914,#93915,#93916,#93917,
#93918,#93919,#93920,#93921,#93922,#93923,#93924,#93925,#93926,#93927,#93928,
#93929,#93930,#93931,#93932,#93933,#93934,#93935,#93936,#93937,#93938,#93939,
#93940,#93941,#93942,#93943,#93944,#93945,#93946,#93947,#93948,#93949,#93950,
#93951,#93952,#93953,#93954,#93955,#93956,#93957,#93958,#93959,#93960,#93961,
#93962,#93963,#93964,#93965,#93966,#93967,#93968,#93969,#93970,#93971,#93972,
#93973,#93974,#93975,#93976,#93977,#93978,#93979,#93980,#93981,#93982,#93983,
#93984,#93985,#93986,#93987,#93988,#93989,#93990,#93991,#93992,#93993,#93994,
#93995,#93996,#93997,#93998,#93999,#94000,#94001,#94002,#94003,#94004,#94005,
#94006,#94007,#94008,#94009,#94010,#94011,#94012,#94013,#94014,#94015,#94016,
#94017,#94018,#94019,#94020,#94021,#94022,#94023,#94024,#94025,#94026,#94027,
#94028,#94029,#94030,#94031,#94032,#94033,#94034,#94035,#94036,#94037,#94038,
#94039,#94040,#94041,#94042,#94043,#94044,#94045,#94046,#94047,#94048,#94049,
#94050,#94051,#94052,#94053,#94054,#94055,#94056,#94057,#94058,#94059,#94060,
#94061,#94062,#94063,#94064,#94065,#94066,#94067,#94068,#94069,#94070,#94071,
#94072,#94073,#94074,#94075,#94076,#94077,#94078,#94079,#94080,#94081,#94082,
#94083,#94084,#94085,#94086,#94087,#94088,#94089,#94090,#94091,#94092,#94093,
#94094,#94095,#94096,#94097,#94098,#94099,#94100,#94101,#94102,#94103,#94104,
#94105,#94106,#94107,#94108,#94109,#94110,#94111,#94112,#94113,#94114,#94115,
#94116,#94117,#94118,#94119,#94120,#94121),.UNSPECIFIED.,.F.,.F.,(4,2,2,
2,2,2,2,2,2,2,2,2,2,2,2,2,2,2,2,2,2,2,2,2,2,2,2,2,2,2,2,2,2,2,2,2,2,2,2,
2,2,2,2,2,2,2,2,2,2,2,2,2,2,2,2,2,2,2,2,2,2,2,2,2,2,2,2,2,2,2,2,2,2,2,2,
2,2,2,2,2,2,2,2,2,2,2,2,2,2,2,2,2,2,2,2,2,2,2,2,2,2,2,2,2,2,2,2,2,2,4),
(-1.40835487559167,-1.37307254520199,-1.33396207472922,-1.33297746517486,
-1.32826978765958,-1.32653031463525,-1.32550498877885,-1.32441215764762,
-1.32290008276663,-1.31930842386976,-1.28016549281244,-1.23134373312473,
-1.22421242156571,-1.22130615748429,-1.21950571749395,-1.21754976684994,
-1.21487491042775,-1.2086415661001,-1.18159630862061,-1.14087068534051,
-1.11820873836828,-1.11535577022776,-1.1139789680588,-1.11290511464636,
-1.11166909773012,-1.10949055300009,-1.09968883730141,-1.05077809615156,
-1.01565733039017,-1.01136167397369,-1.00882015705595,-1.00687922927664,
-1.00480565510356,-1.00155657882795,-0.991244536713203,-0.974681275199111,
-0.941818720452031,-0.928012557124597,-0.921312351597458,-0.905864994709904,
-0.903497100064906,-0.902089524132845,-0.901009368767303,-0.89980591626645,
-0.897774099278516,-0.889883702582577,-0.875166035499657,-0.84610338411909,
-0.803698163326376,-0.799404690588919,-0.796863863675753,-0.794923116069078,
-0.792849398062927,-0.789599393966096,-0.779278480917498,-0.762695330217843,
-0.729817122474957,-0.714522520717224,-0.709793783754855,-0.693941562126337,
-0.69132874945633,-0.68998289233584,-0.688911648318208,-0.687653731154015,
-0.685374419532334,-0.673948879812471,-0.647572481410561,-0.595122290936872,
-0.588188792099026,-0.585315747864345,-0.583521640853107,-0.581561188251501,
-0.57885945895549,-0.572467087930835,-0.526046496549813,-0.484947955450101,
-0.480263099025422,-0.478527317137722,-0.477502866303812,-0.476409862013194,
-0.474895740954519,-0.471290879544853,-0.432950124987159,-0.383317359767356,
-0.376221657164208,-0.373321731259076,-0.371522737828785,-0.369566395509398,
-0.366887460196501,-0.360806573922974,-0.352445743392808,-0.301551263215531,
-0.270313240974031,-0.267401273577692,-0.266013096591154,-0.264938280807216,
-0.263710015850866,-0.261566046808897,-0.252414963614524,-0.203666418748164,
-0.167704289658466,-0.162982355603723,-0.16055955706944,-0.158640675515175,
-0.156487801539827,-0.154258046046508,-0.14661209264506,-0.121083042627241,
-0.100337614168057,-0.0747504804368338),.UNSPECIFIED.);
#938=B_SPLINE_CURVE_WITH_KNOTS('',3,(#94123,#94124,#94125,#94126,#94127,
#94128,#94129,#94130,#94131,#94132,#94133,#94134,#94135,#94136,#94137,#94138,
#94139,#94140,#94141,#94142,#94143,#94144,#94145,#94146,#94147,#94148,#94149,
#94150,#94151,#94152,#94153,#94154,#94155,#94156,#94157,#94158,#94159,#94160,
#94161,#94162,#94163,#94164,#94165,#94166,#94167,#94168,#94169,#94170,#94171,
#94172,#94173,#94174,#94175,#94176,#94177,#94178,#94179,#94180,#94181,#94182,
#94183,#94184,#94185,#94186,#94187,#94188,#94189,#94190,#94191,#94192,#94193,
#94194,#94195,#94196,#94197,#94198,#94199,#94200,#94201,#94202,#94203,#94204,
#94205,#94206,#94207,#94208,#94209,#94210,#94211,#94212,#94213,#94214,#94215,
#94216,#94217,#94218,#94219,#94220,#94221,#94222,#94223,#94224,#94225,#94226,
#94227,#94228,#94229,#94230,#94231,#94232,#94233,#94234,#94235,#94236,#94237,
#94238,#94239,#94240,#94241,#94242,#94243,#94244,#94245,#94246,#94247,#94248,
#94249,#94250,#94251,#94252,#94253,#94254,#94255,#94256,#94257,#94258,#94259,
#94260,#94261,#94262,#94263,#94264,#94265,#94266,#94267,#94268,#94269,#94270,
#94271,#94272,#94273,#94274,#94275,#94276,#94277,#94278,#94279,#94280,#94281,
#94282,#94283,#94284,#94285,#94286,#94287,#94288,#94289,#94290,#94291,#94292,
#94293,#94294,#94295,#94296,#94297,#94298,#94299,#94300,#94301,#94302,#94303),
 .UNSPECIFIED.,.F.,.F.,(4,3,3,3,3,3,3,3,3,3,3,3,3,3,3,3,3,3,3,3,3,3,3,3,
3,3,3,3,3,3,3,3,3,3,3,3,3,3,3,3,3,3,3,3,3,3,3,3,3,3,3,3,3,3,3,3,3,3,3,3,
4),(-104.022525394709,-103.913514251471,-103.878990796035,-103.775596058987,
-103.672354776872,-103.569234811479,-103.46618024327,-103.363157034912,
-103.260131192239,-103.156998425461,-103.053809334051,-102.950437340669,
-102.880154346073,-102.776759609025,-102.67351832691,-102.570398361518,
-102.467343793309,-102.364320584951,-102.261294742278,-102.1581619755,-102.05497288409,
-101.951600890709,-101.881317896111,-101.777923159063,-101.674681876948,
-101.571561911556,-101.468507343347,-101.365484134989,-101.262458292317,
-101.159325525539,-101.056136434129,-100.952764440747,-100.882481446149,
-100.779086709101,-100.675845426986,-100.572725461594,-100.469670893385,
-100.366647685027,-100.263621842355,-100.160489075577,-100.057299984167,
-99.9539279907855,-99.8836449961874,-99.7802502591395,-99.6770089770245,
-99.5738890116322,-99.4708344434233,-99.3678112350656,-99.264785392393,
-99.161652625615,-99.0584635342052,-98.9550915408236,-98.8848085462255,
-98.7829332776307,-98.681193284401,-98.5795525376357,-98.477975149917,-98.3763829554479,
-98.274788368223,-98.1730805291727,-98.0888188327633),.UNSPECIFIED.);
#939=B_SPLINE_CURVE_WITH_KNOTS('',3,(#94304,#94305,#94306,#94307,#94308),
 .UNSPECIFIED.,.F.,.F.,(4,1,4),(-98.0888186411165,-97.8859720962637,-97.7379482602774),
 .UNSPECIFIED.);
#940=B_SPLINE_CURVE_WITH_KNOTS('',3,(#94314,#94315,#94316,#94317,#94318,
#94319,#94320,#94321,#94322,#94323,#94324,#94325,#94326,#94327,#94328,#94329,
#94330,#94331,#94332,#94333,#94334,#94335),.UNSPECIFIED.,.F.,.F.,(4,2,2,
2,2,2,2,2,2,2,4),(-0.0750517120388601,-0.0634020272158219,-0.0604359224018296,
-0.0436144791537637,-0.0399995549168394,-0.0376361167675147,-0.0357225185227288,
-0.0339209992284383,-0.0317709128135895,-0.0286342845934152,-0.000628474799356472),
 .UNSPECIFIED.);
#941=B_SPLINE_CURVE_WITH_KNOTS('',3,(#94336,#94337,#94338,#94339,#94340,
#94341,#94342,#94343,#94344,#94345,#94346,#94347,#94348,#94349,#94350,#94351,
#94352,#94353,#94354,#94355,#94356,#94357,#94358,#94359,#94360,#94361,#94362,
#94363,#94364,#94365,#94366,#94367,#94368,#94369,#94370,#94371,#94372,#94373,
#94374,#94375,#94376,#94377,#94378,#94379,#94380,#94381,#94382,#94383,#94384,
#94385,#94386,#94387,#94388,#94389,#94390,#94391,#94392,#94393,#94394,#94395,
#94396,#94397,#94398,#94399,#94400,#94401,#94402,#94403,#94404,#94405,#94406,
#94407,#94408,#94409,#94410,#94411,#94412,#94413,#94414,#94415,#94416,#94417,
#94418,#94419,#94420,#94421,#94422,#94423,#94424,#94425,#94426,#94427,#94428,
#94429,#94430,#94431,#94432,#94433,#94434,#94435,#94436,#94437,#94438,#94439,
#94440,#94441,#94442,#94443,#94444,#94445,#94446,#94447,#94448,#94449,#94450,
#94451,#94452,#94453,#94454,#94455,#94456,#94457,#94458,#94459,#94460,#94461,
#94462,#94463,#94464,#94465,#94466,#94467,#94468,#94469,#94470,#94471,#94472,
#94473,#94474,#94475,#94476,#94477,#94478,#94479,#94480,#94481,#94482,#94483,
#94484,#94485,#94486,#94487,#94488,#94489,#94490,#94491,#94492,#94493,#94494,
#94495,#94496,#94497,#94498,#94499,#94500,#94501,#94502,#94503,#94504,#94505,
#94506,#94507,#94508,#94509,#94510,#94511,#94512,#94513,#94514,#94515,#94516,
#94517,#94518,#94519,#94520,#94521,#94522,#94523,#94524,#94525,#94526,#94527,
#94528,#94529,#94530,#94531,#94532,#94533,#94534,#94535,#94536,#94537,#94538,
#94539,#94540,#94541,#94542,#94543,#94544,#94545,#94546,#94547,#94548,#94549,
#94550,#94551,#94552,#94553,#94554,#94555,#94556,#94557),.UNSPECIFIED.,
 .F.,.F.,(4,2,2,2,2,2,2,2,2,2,2,2,2,2,2,2,2,2,2,2,2,2,2,2,2,2,2,2,2,2,2,
2,2,2,2,2,2,2,2,2,2,2,2,2,2,2,2,2,2,2,2,2,2,2,2,2,2,2,2,2,2,2,2,2,2,2,2,
2,2,2,2,2,2,2,2,2,2,2,2,2,2,2,2,2,2,2,2,2,2,2,2,2,2,2,2,2,2,2,2,2,2,2,2,
2,2,2,2,2,2,2,4),(-2.66763698055154,-2.62406132926978,-2.60408125324982,
-2.60008719792512,-2.59850914862046,-2.59740414699734,-2.59639472646751,
-2.59473746711411,-2.59055157721239,-2.5405210743688,-2.51637322760607,
-2.50454754215916,-2.49656808709728,-2.49362515114192,-2.49183396792167,
-2.48989323829761,-2.48735333064289,-2.4830634488436,-2.44793672455365,
-2.39902535700703,-2.38925433004982,-2.38707788654155,-2.38584232285153,
-2.38476839530661,-2.38339087700578,-2.38053430428018,-2.35748862309685,
-2.31189038376125,-2.28922915612821,-2.2835614525403,-2.28098732924355,
-2.27904817786268,-2.27722187816149,-2.27468221218954,-2.26805709348043,
-2.21208953581673,-2.18811951732637,-2.1773202970419,-2.17507749882885,
-2.17382737629828,-2.17275518583563,-2.17139841206732,-2.1692508923137,
-2.1581870041224,-2.10689039676946,-2.07825808558725,-2.07183293481812,
-2.06912537405989,-2.06716360905802,-2.06537031487206,-2.06250294852276,
-2.05560575299052,-2.00267094463175,-1.97665318563582,-1.96531689598131,
-1.96304242698115,-1.96178542969317,-1.96071390982458,-1.95936635215361,
-1.95674626440744,-1.94073469003329,-1.93573867539908,-1.93132393603383,
-1.89233935142684,-1.86585640669193,-1.85969308426041,-1.85703032509592,
-1.85507646846316,-1.85327322083275,-1.85035184993496,-1.8431307686578,
-1.79858280033235,-1.78473559685624,-1.76327650800007,-1.75318374826895,
-1.75098568762849,-1.74974536357142,-1.7486720627611,-1.74730154345496,
-1.74510875810344,-1.7333397544113,-1.72962685146761,-1.72236555834075,
-1.67901009052207,-1.66042268314643,-1.6492198747353,-1.64587221252619,
-1.64377679847104,-1.64184352623183,-1.63935164536473,-1.6352264317297,
-1.60809055958966,-1.56616636875005,-1.54954736470946,-1.54098478387904,
-1.53889723321266,-1.53768129423243,-1.53660390200266,-1.53521797705394,
-1.53292427051012,-1.51915032158516,-1.50784480255644,-1.46844818274825,
-1.44187537801273,-1.43570086543967,-1.43303615705244,-1.43108195608314,
-1.42927915315622,-1.42636020630751,-1.41915354224474,-1.40835487559167),
 .UNSPECIFIED.);
#942=B_SPLINE_CURVE_WITH_KNOTS('',3,(#94559,#94560,#94561,#94562,#94563,
#94564,#94565,#94566,#94567,#94568),.UNSPECIFIED.,.F.,.F.,(4,1,1,1,1,1,
1,4),(-97.7379482602774,-96.8871356463018,-95.8882991963399,-94.889462746378,
-93.8906262964162,-92.8917898464543,-91.8929533964924,-91.8056333339369),
 .UNSPECIFIED.);
#943=B_SPLINE_CURVE_WITH_KNOTS('',3,(#94569,#94570,#94571,#94572,#94573,
#94574,#94575,#94576),.UNSPECIFIED.,.F.,.F.,(4,2,2,4),(-2.66772514762063,
-2.61547416970725,-2.59711068312006,-2.59328853658183),.UNSPECIFIED.);
#944=B_SPLINE_CURVE_WITH_KNOTS('',3,(#94581,#94582,#94583,#94584,#94585,
#94586,#94587,#94588,#94589,#94590,#94591,#94592,#94593,#94594,#94595,#94596,
#94597,#94598,#94599,#94600,#94601,#94602,#94603,#94604,#94605,#94606,#94607,
#94608,#94609,#94610,#94611,#94612,#94613,#94614,#94615,#94616,#94617,#94618,
#94619,#94620,#94621,#94622,#94623,#94624,#94625,#94626,#94627,#94628,#94629,
#94630,#94631,#94632,#94633,#94634,#94635,#94636,#94637,#94638,#94639,#94640,
#94641,#94642,#94643,#94644,#94645,#94646,#94647,#94648,#94649,#94650,#94651,
#94652,#94653,#94654,#94655,#94656,#94657,#94658,#94659,#94660,#94661,#94662,
#94663,#94664,#94665,#94666,#94667,#94668,#94669,#94670,#94671,#94672,#94673,
#94674,#94675,#94676,#94677,#94678,#94679,#94680,#94681,#94682,#94683,#94684,
#94685,#94686,#94687,#94688,#94689,#94690,#94691,#94692,#94693,#94694,#94695,
#94696,#94697,#94698,#94699,#94700,#94701,#94702,#94703,#94704,#94705,#94706,
#94707,#94708,#94709,#94710,#94711,#94712,#94713,#94714,#94715,#94716,#94717,
#94718,#94719,#94720,#94721,#94722,#94723,#94724,#94725,#94726,#94727,#94728,
#94729,#94730,#94731,#94732,#94733,#94734,#94735,#94736,#94737,#94738,#94739,
#94740,#94741,#94742,#94743,#94744,#94745,#94746,#94747,#94748,#94749,#94750,
#94751,#94752,#94753,#94754,#94755,#94756,#94757,#94758,#94759,#94760,#94761,
#94762,#94763,#94764,#94765,#94766,#94767,#94768,#94769,#94770,#94771,#94772,
#94773,#94774,#94775,#94776,#94777,#94778,#94779,#94780,#94781,#94782,#94783,
#94784,#94785,#94786,#94787,#94788,#94789,#94790,#94791,#94792,#94793,#94794,
#94795,#94796),.UNSPECIFIED.,.F.,.F.,(4,2,2,2,2,2,2,2,2,2,2,2,2,2,2,2,2,
2,2,2,2,2,2,2,2,2,2,2,2,2,2,2,2,2,2,2,2,2,2,2,2,2,2,2,2,2,2,2,2,2,2,2,2,
2,2,2,2,2,2,2,2,2,2,2,2,2,2,2,2,2,2,2,2,2,2,2,2,2,2,2,2,2,2,2,2,2,2,2,2,
2,2,2,2,2,2,2,2,2,2,2,2,2,2,2,2,2,2,4),(-1.40856923606383,-1.37753534771955,
-1.33437657332176,-1.31573891594647,-1.3120061968455,-1.30960628755538,
-1.30768951854701,-1.30552196583,-1.30184736841551,-1.28708445286655,-1.25915940004959,
-1.20936248341951,-1.20515952976254,-1.20349955493878,-1.20248976234215,
-1.20138551989213,-1.19981053362183,-1.19583462843233,-1.17602196558166,
-1.14710916065381,-1.10479021809735,-1.10049510372887,-1.09795386327688,
-1.09601312115518,-1.09393972062583,-1.09069086485238,-1.08037908770372,
-1.06381583815358,-1.03095505388635,-1.01702991026295,-1.01060149811018,
-0.99501784778292,-0.992416272356635,-0.99107287879295,-0.990001836063541,
-0.988742108789686,-0.986454280833403,-0.974876064563483,-0.947886078247631,
-0.896303554775745,-0.889312743805389,-0.886430318131219,-0.884634560714498,
-0.882675665973707,-0.879982209663275,-0.873638078681677,-0.845678864518596,
-0.799178081163946,-0.783068285307751,-0.780441711403226,-0.77909295100005,
-0.778021593748141,-0.776766088572937,-0.774497609916402,-0.763258791406917,
-0.737615135793081,-0.684120852360988,-0.677267512448455,-0.674407789435915,
-0.672616199818987,-0.670653827861174,-0.667940880716456,-0.661481313481932,
-0.607554754257518,-0.571347485437789,-0.568493308914977,-0.567116455231962,
-0.566042811664781,-0.564807318673821,-0.56263037346325,-0.552847073374781,
-0.503933837770377,-0.468823844809091,-0.464525049280988,-0.461982917923506,
-0.460042236207826,-0.457969618093723,-0.454723486350996,-0.444432967339147,
-0.427915840221092,-0.371222029924013,-0.358723107565275,-0.356494168675288,
-0.355112906516237,-0.354038846722208,-0.352806275989511,-0.350642575110138,
-0.341050887842663,-0.2919753618443,-0.256812359758064,-0.252513848206065,
-0.249971815109268,-0.248031168310692,-0.246240519153969,-0.243303174156408,
-0.235328939247043,-0.223525724651994,-0.190999540386583,-0.150078407977255,
-0.145387637847395,-0.143651113117761,-0.142626620365515,-0.141533908489056,
-0.140020743226501,-0.136420702779226,-0.0985274263552539,-0.0757357778527809,
-0.0750517120388601),.UNSPECIFIED.);
#945=B_SPLINE_CURVE_WITH_KNOTS('',3,(#94797,#94798,#94799,#94800,#94801,
#94802,#94803,#94804,#94805,#94806,#94807,#94808,#94809,#94810,#94811,#94812,
#94813,#94814,#94815,#94816,#94817,#94818,#94819,#94820,#94821,#94822,#94823,
#94824,#94825,#94826,#94827,#94828,#94829,#94830,#94831,#94832,#94833,#94834,
#94835,#94836,#94837,#94838,#94839,#94840,#94841,#94842,#94843,#94844,#94845,
#94846,#94847,#94848,#94849,#94850,#94851,#94852,#94853,#94854,#94855,#94856,
#94857,#94858,#94859,#94860,#94861,#94862,#94863,#94864,#94865,#94866,#94867,
#94868,#94869,#94870,#94871,#94872,#94873,#94874,#94875,#94876,#94877,#94878,
#94879,#94880,#94881,#94882,#94883,#94884,#94885,#94886,#94887,#94888,#94889,
#94890,#94891,#94892,#94893,#94894,#94895,#94896,#94897,#94898,#94899,#94900,
#94901,#94902,#94903,#94904,#94905,#94906,#94907,#94908,#94909,#94910,#94911,
#94912,#94913,#94914,#94915,#94916,#94917,#94918,#94919,#94920,#94921,#94922,
#94923,#94924,#94925,#94926,#94927,#94928,#94929,#94930,#94931,#94932,#94933,
#94934,#94935,#94936,#94937,#94938,#94939,#94940,#94941,#94942,#94943,#94944,
#94945,#94946,#94947,#94948,#94949,#94950,#94951,#94952,#94953,#94954,#94955,
#94956,#94957,#94958,#94959,#94960,#94961,#94962,#94963,#94964,#94965,#94966,
#94967,#94968,#94969,#94970,#94971,#94972,#94973,#94974,#94975,#94976,#94977,
#94978,#94979,#94980,#94981,#94982,#94983,#94984,#94985,#94986,#94987,#94988,
#94989,#94990,#94991,#94992,#94993,#94994,#94995,#94996,#94997,#94998,#94999,
#95000,#95001,#95002,#95003,#95004,#95005,#95006,#95007,#95008,#95009,#95010,
#95011,#95012,#95013,#95014,#95015,#95016,#95017,#95018,#95019,#95020,#95021,
#95022,#95023,#95024,#95025,#95026,#95027,#95028,#95029,#95030,#95031,#95032,
#95033,#95034,#95035,#95036,#95037,#95038,#95039,#95040,#95041,#95042,#95043,
#95044,#95045,#95046,#95047,#95048,#95049,#95050,#95051,#95052,#95053,#95054,
#95055,#95056,#95057,#95058,#95059,#95060,#95061,#95062,#95063,#95064,#95065,
#95066,#95067,#95068,#95069,#95070),.UNSPECIFIED.,.F.,.F.,(4,2,2,2,2,2,
2,2,2,2,2,2,2,2,2,2,2,2,2,2,2,2,2,2,2,2,2,2,2,2,2,2,2,2,2,2,2,2,2,2,2,2,
2,2,2,2,2,2,2,2,2,2,2,2,2,2,2,2,2,2,2,2,2,2,2,2,2,2,2,2,2,2,2,2,2,2,2,2,
2,2,2,2,2,2,2,2,2,2,2,2,2,2,2,2,2,2,2,2,2,2,2,2,2,2,2,2,2,2,2,2,2,2,2,2,
2,2,2,2,2,2,2,2,2,2,2,2,2,2,2,2,2,2,2,2,2,2,4),(-2.59328853658183,-2.58600535494844,
-2.58266887539578,-2.58057642818646,-2.57864314721145,-2.57614740908341,
-2.57200747303872,-2.54425453014782,-2.50200628554234,-2.48610512911484,
-2.48058315091995,-2.47794773478339,-2.47583510493174,-2.47461246849111,
-2.47460891636769,-2.47460535047061,-2.47460177083311,-2.47459817731066,
-2.4745943200395,-2.47459039557256,-2.47458640246708,-2.47458233940881,
-2.47457820487136,-2.4745739972196,-2.47456971496081,-2.47456535648725,
-2.47456092015516,-2.47455640412381,-2.47455180666171,-2.47454712608477,
-2.47454236042841,-2.47453750779661,-2.47351268581807,-2.47213899916749,
-2.46930049460154,-2.43223374368189,-2.40047018286322,-2.37797733684563,
-2.37233324391901,-2.36976395145162,-2.36782603975058,-2.36599914366965,
-2.36345581671894,-2.35680429041609,-2.30111490358013,-2.27698401532335,
-2.26614276803842,-2.26389793128162,-2.262647608935,-2.26157582430046,-2.26022030442467,
-2.25807615650924,-2.24705912450343,-2.19580516494524,-2.16711833686923,
-2.16068765539593,-2.15797968196895,-2.15601831413085,-2.15422586190681,
-2.1513608837026,-2.14447482915395,-2.09143998963289,-2.0655120480464,-2.05420013507617,
-2.05192758608789,-2.05067125065163,-2.04960005262515,-2.04825259117729,
-2.04563178322568,-2.02959904215348,-2.02426125641956,-2.00971680617145,
-1.97682916778035,-1.9602647611674,-1.9499537921242,-1.94670523996688,-1.94463205138889,
-1.94269152097581,-1.94015057817655,-1.93585604478312,-1.90074428505616,
-1.85183366806679,-1.84207811610761,-1.83990309602701,-1.8386680283493,
-1.83759433212019,-1.83621684929797,-1.83335945110605,-1.81024465379414,
-1.76802196894324,-1.74940024809552,-1.7381835766657,-1.73483500762019,
-1.73273974756283,-1.73080710725478,-1.72831672515025,-1.72419547147613,
-1.69718015320056,-1.65528661855897,-1.63857253188948,-1.62997826973702,
-1.62788858529347,-1.62667237010685,-1.62559538417855,-1.62421082132829,
-1.62192110600651,-1.60822077698475,-1.6063709175413,-1.60500956888155,
-1.59754429260797,-1.5857463123036,-1.55288290217087,-1.53634916327188,
-1.52605188241343,-1.52280476620983,-1.52073180221146,-1.51879099585163,
-1.51624899004895,-1.51195108676669,-1.47659208805181,-1.42743052032568,
-1.41811510554275,-1.41597092291642,-1.41474259634102,-1.41366777160722,
-1.41227963173231,-1.40936793125375,-1.37753518125494,-1.33437642004195,
-1.3157387709112,-1.31200605408965,-1.30960614637965,-1.30768937871047,
-1.30552182759218,-1.30184723310008,-1.28708433244916,-1.2599708008188),
 .UNSPECIFIED.);
#946=B_SPLINE_CURVE_WITH_KNOTS('',3,(#95076,#95077,#95078,#95079,#95080),
 .UNSPECIFIED.,.F.,.F.,(4,1,4),(82.6397394568681,82.9034253468356,82.9907454093913),
 .UNSPECIFIED.);
#947=B_SPLINE_CURVE_WITH_KNOTS('',3,(#95081,#95082,#95083,#95084,#95085,
#95086,#95087,#95088,#95089,#95090,#95091,#95092,#95093,#95094,#95095,#95096,
#95097,#95098,#95099,#95100,#95101,#95102,#95103,#95104,#95105,#95106,#95107,
#95108,#95109,#95110,#95111,#95112,#95113,#95114,#95115,#95116,#95117,#95118,
#95119,#95120,#95121,#95122,#95123,#95124,#95125,#95126,#95127,#95128,#95129,
#95130,#95131,#95132,#95133,#95134,#95135,#95136,#95137,#95138,#95139,#95140,
#95141,#95142,#95143,#95144,#95145,#95146,#95147,#95148,#95149,#95150,#95151,
#95152,#95153,#95154,#95155,#95156,#95157,#95158,#95159,#95160,#95161,#95162,
#95163,#95164,#95165,#95166,#95167,#95168,#95169,#95170,#95171,#95172,#95173,
#95174,#95175,#95176,#95177,#95178,#95179,#95180,#95181,#95182,#95183,#95184,
#95185,#95186,#95187,#95188,#95189,#95190,#95191,#95192,#95193,#95194,#95195,
#95196,#95197,#95198,#95199,#95200,#95201,#95202,#95203,#95204,#95205,#95206,
#95207,#95208,#95209,#95210,#95211,#95212,#95213,#95214,#95215,#95216,#95217,
#95218,#95219,#95220,#95221,#95222,#95223,#95224,#95225,#95226,#95227,#95228,
#95229,#95230,#95231,#95232,#95233,#95234,#95235,#95236,#95237,#95238,#95239,
#95240,#95241,#95242,#95243,#95244,#95245,#95246,#95247,#95248,#95249,#95250,
#95251,#95252,#95253,#95254,#95255,#95256,#95257,#95258,#95259,#95260,#95261,
#95262,#95263,#95264,#95265,#95266,#95267,#95268,#95269,#95270,#95271,#95272,
#95273,#95274,#95275,#95276,#95277,#95278,#95279,#95280,#95281,#95282,#95283,
#95284,#95285,#95286,#95287,#95288,#95289,#95290,#95291,#95292,#95293,#95294,
#95295,#95296,#95297,#95298,#95299,#95300,#95301,#95302,#95303,#95304,#95305,
#95306,#95307,#95308,#95309,#95310,#95311,#95312,#95313,#95314,#95315,#95316,
#95317,#95318,#95319,#95320,#95321,#95322,#95323,#95324,#95325,#95326,#95327,
#95328,#95329,#95330,#95331,#95332,#95333,#95334,#95335,#95336),
 .UNSPECIFIED.,.F.,.F.,(4,2,2,2,2,2,2,2,2,2,2,2,2,2,2,2,2,2,2,2,2,2,2,2,
2,2,2,2,2,2,2,2,2,2,2,2,2,2,2,2,2,2,2,2,2,2,2,2,2,2,2,2,2,2,2,2,2,2,2,2,
2,2,2,2,2,2,2,2,2,2,2,2,2,2,2,2,2,2,2,2,2,2,2,2,2,2,2,2,2,2,2,2,2,2,2,2,
2,2,2,2,2,2,2,2,2,2,2,2,2,2,2,2,2,2,2,2,2,2,2,2,2,2,2,2,2,2,2,4),(-2.66780040318838,
-2.61551790977789,-2.59716970564285,-2.58607064758385,-2.58273462170918,
-2.58064213716017,-2.57870860232032,-2.57621222890874,-2.57207057156959,
-2.54426538375466,-2.50203381017613,-2.48615303607179,-2.48063557805295,
-2.4780016315159,-2.47588992400724,-2.47466741989728,-2.47466386489016,
-2.47466029622126,-2.47465671365226,-2.47465311723954,-2.47464924790979,
-2.4746453111953,-2.47464130566459,-2.47463722980043,-2.4746330821842,-2.47462886123928,
-2.47462456548351,-2.47462019315263,-2.4746157426227,-2.47461121211173,
-2.47460659981634,-2.47460190392262,-2.47459712275845,-2.47459225433639,
-2.47356702128603,-2.47219259175844,-2.46935060110709,-2.43244643100335,
-2.40084454662119,-2.38427063419762,-2.37395535867637,-2.37070630606194,
-2.36863300375729,-2.36669251132516,-2.36415182660582,-2.35985819626608,
-2.32481492744113,-2.27610713395617,-2.26610865268452,-2.26391722830508,
-2.26267855532423,-2.26160535599814,-2.2602332393536,-2.25740312238981,
-2.23560475967612,-2.19422095111495,-2.16695271661404,-2.16069314305251,
-2.15801416376571,-2.15605785333276,-2.15425893775005,-2.15135923276972,
-2.14426456299575,-2.0946777819443,-2.05630537544114,-2.05272022306183,
-2.05120950165274,-2.05011712916657,-2.04909182103223,-2.04735149707135,
-2.04263638471332,-2.00208399405331,-1.95512537277313,-1.94873124009659,
-1.9460293282421,-1.94406895064217,-1.94227505926827,-1.93940266956448,
-1.93247232764485,-1.88002504947992,-1.85368147982009,-1.84226394811427,
-1.83998524791738,-1.83872752180653,-1.83765635537541,-1.83631048147007,
-1.83369730300961,-1.81782808212738,-1.81196103643523,-1.76792203456759,
-1.74936661043314,-1.73817836764796,-1.73483281711261,-1.73273822411008,
-1.73080536922593,-1.72831355082763,-1.72418741219789,-1.69698007334459,
-1.65492989181173,-1.63847229080999,-1.62996575863749,-1.62788302762729,
-1.62666835416131,-1.6255910415935,-1.62420387356723,-1.62190531774929,
-1.608022288628,-1.60651774343736,-1.60499935810568,-1.59754569688297,-1.5857466200268,
-1.55288318433354,-1.53634942709176,-1.52605213609457,-1.52280501728472,
-1.52073205175766,-1.51879124405963,-1.51624923663557,-1.51195133089639,
-1.47659233779622,-1.42743072687935,-1.41811530320247,-1.41597111890691,
-1.41474279143201,-1.41366796594469,-1.41227982512901,-1.40936812278207,
-1.40856923606383),.UNSPECIFIED.);
#948=B_SPLINE_CURVE_WITH_KNOTS('',3,(#95338,#95339,#95340,#95341,#95342,
#95343,#95344,#95345,#95346,#95347,#95348,#95349,#95350,#95351,#95352,#95353,
#95354,#95355,#95356,#95357,#95358,#95359,#95360,#95361,#95362,#95363,#95364,
#95365,#95366,#95367,#95368,#95369,#95370,#95371,#95372,#95373,#95374,#95375,
#95376,#95377,#95378,#95379,#95380,#95381,#95382,#95383,#95384,#95385,#95386,
#95387,#95388,#95389,#95390,#95391,#95392,#95393,#95394,#95395,#95396,#95397,
#95398,#95399,#95400,#95401,#95402,#95403,#95404,#95405,#95406,#95407,#95408,
#95409,#95410,#95411,#95412,#95413,#95414,#95415,#95416,#95417,#95418,#95419,
#95420,#95421,#95422,#95423,#95424,#95425,#95426,#95427,#95428,#95429,#95430,
#95431,#95432,#95433,#95434,#95435,#95436,#95437,#95438,#95439,#95440,#95441,
#95442,#95443,#95444,#95445,#95446,#95447,#95448,#95449,#95450,#95451,#95452,
#95453,#95454,#95455,#95456,#95457,#95458,#95459,#95460,#95461,#95462,#95463,
#95464,#95465,#95466,#95467,#95468,#95469,#95470,#95471,#95472,#95473,#95474,
#95475,#95476,#95477,#95478,#95479,#95480,#95481,#95482,#95483,#95484,#95485,
#95486,#95487,#95488,#95489,#95490,#95491,#95492,#95493,#95494,#95495,#95496,
#95497,#95498,#95499,#95500,#95501,#95502,#95503,#95504,#95505,#95506,#95507,
#95508,#95509,#95510,#95511,#95512,#95513,#95514,#95515,#95516,#95517,#95518,
#95519,#95520,#95521,#95522,#95523,#95524,#95525,#95526,#95527,#95528,#95529,
#95530,#95531,#95532,#95533,#95534,#95535,#95536,#95537,#95538,#95539,#95540,
#95541,#95542,#95543,#95544,#95545,#95546,#95547,#95548,#95549,#95550,#95551,
#95552,#95553),.UNSPECIFIED.,.F.,.F.,(4,2,2,2,2,2,2,2,2,2,2,2,2,2,2,2,2,
2,2,2,2,2,2,2,2,2,2,2,2,2,2,2,2,2,2,2,2,2,2,2,2,2,2,2,2,2,2,2,2,2,2,2,2,
2,2,2,2,2,2,2,2,2,2,2,2,2,2,2,2,2,2,2,2,2,2,2,2,2,2,2,2,2,2,2,2,2,2,2,2,
2,2,2,2,2,2,2,2,2,2,2,2,2,2,2,2,2,2,4),(-1.2599708008188,-1.25915931404613,
-1.2093623898908,-1.20515944082174,-1.20349946744209,-1.2024896756088,-1.20138543389462,
-1.19981044851553,-1.1958345447609,-1.17602188346793,-1.14710909938688,
-1.10479018083132,-1.10049506909096,-1.09795383031137,-1.09601308953707,
-1.09393969051777,-1.09069083726277,-1.08037906948267,-1.06381583657343,
-1.03095507642963,-1.01703064325082,-1.01060069523947,-0.99501781415168,
-0.992416272899047,-0.991072887307461,-0.990001845800765,-0.988742114004146,
-0.986454262563982,-0.974875604050108,-0.947883813621921,-0.896303853404042,
-0.88931288873904,-0.886430438880445,-0.884634677984654,-0.882675788698833,
-0.879982356728087,-0.873638361634836,-0.845680254375092,-0.799190303148751,
-0.783069938021953,-0.780442462190926,-0.779093508375728,-0.778022138915881,
-0.776766783138712,-0.774498989100002,-0.763271961099305,-0.737674112670588,
-0.684113440102638,-0.677265491733396,-0.674406658048039,-0.672615230367634,
-0.67065271711738,-0.667938988470744,-0.661474766328608,-0.607387867162281,
-0.571356310839664,-0.56849630893015,-0.567118312414115,-0.566044560387861,
-0.564809825832879,-0.562636327992937,-0.552903371534513,-0.503947647622929,
-0.468806965956647,-0.464517412680411,-0.461977961282968,-0.460037720253713,
-0.457964015604134,-0.45471292912842,-0.444379256455963,-0.427766718973355,
-0.371066935348685,-0.35870882090716,-0.356487415483326,-0.355108425874969,
-0.354034588942138,-0.352800533488199,-0.350630083729614,-0.34094115553311,
-0.291948731762867,-0.256811880824043,-0.252513633573081,-0.249971677306362,
-0.248031043426507,-0.246240395005676,-0.243302955670095,-0.235328059303593,
-0.223523564485029,-0.190998708291966,-0.150078465375664,-0.145387649929409,
-0.143651118521622,-0.142626624597578,-0.141533913829228,-0.140020753964473,
-0.136420744214609,-0.0985305953414833,-0.0757357801255632,-0.0634020321071917,
-0.0604357409625306,-0.0436144588626216,-0.0399995457881178,-0.0376361113317291,
-0.0357225136846189,-0.0339209943472396,-0.0317709061040813,-0.0286342730469093,
-0.000628476936311304),.UNSPECIFIED.);
#949=B_SPLINE_CURVE_WITH_KNOTS('',3,(#95554,#95555,#95556,#95557,#95558,
#95559,#95560,#95561,#95562,#95563,#95564,#95565,#95566,#95567,#95568,#95569,
#95570,#95571),.UNSPECIFIED.,.F.,.F.,(4,2,2,2,2,2,2,2,4),(-2.66755959603529,
-2.62120144362155,-2.60363571981804,-2.59990254938237,-2.59836672373323,
-2.59726968673265,-2.59625060032127,-2.59454299008746,-2.59340588318677),
 .UNSPECIFIED.);
#950=B_SPLINE_CURVE_WITH_KNOTS('',3,(#95577,#95578,#95579,#95580,#95581,
#95582,#95583,#95584,#95585,#95586,#95587,#95588,#95589),.UNSPECIFIED.,
 .F.,.F.,(4,3,3,3,4),(76.3573194351122,76.4589087580869,76.5605127537386,
76.6622237693788,76.7075599105176),.UNSPECIFIED.);
#951=B_SPLINE_CURVE_WITH_KNOTS('',3,(#95590,#95591,#95592,#95593,#95594,
#95595,#95596,#95597,#95598,#95599),.UNSPECIFIED.,.F.,.F.,(4,1,1,1,1,1,
1,4),(76.7075601022117,76.9104066470643,77.9092430970262,78.9080795469881,
79.9069159969499,80.9057524469118,81.9045888968737,82.6397394568681),
 .UNSPECIFIED.);
#952=B_SPLINE_CURVE_WITH_KNOTS('',3,(#95600,#95601,#95602,#95603,#95604,
#95605,#95606,#95607,#95608,#95609,#95610,#95611,#95612,#95613,#95614,#95615,
#95616,#95617,#95618,#95619,#95620,#95621,#95622,#95623,#95624,#95625,#95626,
#95627,#95628,#95629,#95630,#95631,#95632,#95633,#95634,#95635,#95636,#95637,
#95638,#95639,#95640,#95641,#95642,#95643,#95644,#95645,#95646,#95647,#95648,
#95649,#95650,#95651,#95652,#95653,#95654,#95655,#95656,#95657,#95658,#95659,
#95660,#95661,#95662,#95663,#95664,#95665,#95666,#95667,#95668,#95669,#95670,
#95671,#95672,#95673,#95674,#95675,#95676,#95677,#95678,#95679,#95680,#95681,
#95682,#95683,#95684,#95685,#95686,#95687,#95688,#95689,#95690,#95691,#95692,
#95693,#95694,#95695,#95696,#95697,#95698,#95699,#95700,#95701,#95702,#95703,
#95704,#95705,#95706,#95707,#95708,#95709,#95710,#95711,#95712,#95713,#95714,
#95715,#95716,#95717,#95718,#95719,#95720,#95721,#95722,#95723,#95724,#95725,
#95726,#95727,#95728,#95729,#95730,#95731,#95732,#95733,#95734,#95735,#95736,
#95737,#95738,#95739,#95740,#95741,#95742,#95743,#95744,#95745,#95746,#95747,
#95748,#95749,#95750,#95751,#95752,#95753,#95754,#95755,#95756,#95757,#95758,
#95759,#95760,#95761,#95762,#95763,#95764,#95765,#95766,#95767,#95768,#95769,
#95770,#95771,#95772,#95773,#95774,#95775,#95776,#95777,#95778,#95779,#95780,
#95781,#95782,#95783,#95784,#95785,#95786,#95787,#95788,#95789,#95790,#95791,
#95792,#95793,#95794,#95795,#95796,#95797,#95798,#95799,#95800,#95801,#95802,
#95803,#95804,#95805,#95806,#95807,#95808,#95809,#95810,#95811,#95812,#95813,
#95814,#95815,#95816,#95817,#95818,#95819,#95820,#95821,#95822,#95823,#95824,
#95825,#95826,#95827,#95828,#95829,#95830,#95831,#95832,#95833,#95834,#95835),
 .UNSPECIFIED.,.F.,.F.,(4,2,2,2,2,2,2,2,2,2,2,2,2,2,2,2,2,2,2,2,2,2,2,2,
2,2,2,2,2,2,2,2,2,2,2,2,2,2,2,2,2,2,2,2,2,2,2,2,2,2,2,2,2,2,2,2,2,2,2,2,
2,2,2,2,2,2,2,2,2,2,2,2,2,2,2,2,2,2,2,2,2,2,2,2,2,2,2,2,2,2,2,2,2,2,2,2,
2,2,2,2,2,2,2,2,2,2,2,2,2,2,2,2,2,2,2,2,2,4),(-2.59340588318677,-2.59004423660487,
-2.54306658858682,-2.5229269865908,-2.50702016726606,-2.50036241947781,
-2.4952935381366,-2.49283512899737,-2.49090555118735,-2.48905817955765,
-2.48590554168906,-2.47720771247942,-2.47623867732846,-2.42660023042714,
-2.40067333012771,-2.3893602005497,-2.38708707027063,-2.38583036818752,
-2.38475883004618,-2.38341090575629,-2.38078909458786,-2.36474844614091,
-2.35942605859247,-2.31445345040613,-2.29625802577929,-2.28522426279168,
-2.28189473509369,-2.27980335788013,-2.27786881899704,-2.27536830200985,
-2.27121357898737,-2.24314199458864,-2.20093986094052,-2.18522736912133,
-2.17697939416692,-2.17491728352695,-2.17370700818838,-2.17262838938498,
-2.17123277416945,-2.16890605074208,-2.15452038519105,-2.15352883894173,
-2.10778334801586,-2.07838985863533,-2.07187460704002,-2.06915190389629,
-2.06718737487783,-2.06539717179839,-2.06254690361088,-2.05575334937012,
-2.00154684777688,-1.9764045095012,-1.96529377242664,-1.96303239086358,
-1.96177823745429,-1.9607064650167,-1.95935517262548,-1.95671772526564,
-1.9402748759459,-1.93129636558274,-1.89233352323295,-1.86585502833783,
-1.85969225800642,-1.85702959369709,-1.85507575252038,-1.85327248110821,
-1.85035098660948,-1.84312917975894,-1.79882622206036,-1.78472750953159,
-1.76327452968949,-1.75318355692263,-1.75098561428941,-1.74974531626441,
-1.74867201233729,-1.74730145574685,-1.7451085468767,-1.73333762184774,
-1.72962677687866,-1.72236564285951,-1.67901010698359,-1.66042270102561,
-1.64921989367379,-1.64587223199068,-1.64377681831943,-1.64184354647315,
-1.63935166617003,-1.63522645360109,-1.60809060278197,-1.56616641224731,
-1.54954739102426,-1.54098480469842,-1.53889725386835,-1.5376813150003,
-1.53660392301353,-1.53521799857436,-1.53292429328767,-1.51915036422728,
-1.50784474804067,-1.46844818562436,-1.44187539553467,-1.43570088525707,
-1.43303617757835,-1.43108197702624,-1.42927917441425,-1.4263602279219,
-1.41915356401649,-1.3730725829945,-1.33396209695869,-1.33297754939684,
-1.32826982446248,-1.32653034444181,-1.32550501734818,-1.32441218735223,
-1.32290011805811,-1.3193084909293,-1.28017013564396,-1.2596844006188),
 .UNSPECIFIED.);
#953=B_SPLINE_CURVE_WITH_KNOTS('',3,(#95841,#95842,#95843,#95844,#95845,
#95846,#95847,#95848,#95849,#95850,#95851,#95852,#95853,#95854,#95855,#95856,
#95857,#95858),.UNSPECIFIED.,.F.,.F.,(4,2,2,2,2,2,2,2,4),(-0.0749220714811919,
-0.0643002951613714,-0.0267279186973627,-0.018764011404856,-0.00802108956177915,
-0.0046663291600887,-0.00258130050280219,-0.00128118356189532,-0.000628940416801203),
 .UNSPECIFIED.);
#954=B_SPLINE_CURVE_WITH_KNOTS('',3,(#95859,#95860,#95861,#95862,#95863,
#95864,#95865,#95866,#95867,#95868,#95869,#95870,#95871,#95872,#95873,#95874,
#95875,#95876,#95877,#95878,#95879,#95880,#95881,#95882,#95883,#95884,#95885,
#95886,#95887,#95888,#95889,#95890,#95891,#95892,#95893,#95894,#95895,#95896,
#95897,#95898,#95899,#95900,#95901,#95902,#95903,#95904,#95905,#95906,#95907,
#95908,#95909,#95910,#95911,#95912,#95913,#95914,#95915,#95916,#95917,#95918,
#95919,#95920,#95921,#95922,#95923,#95924,#95925,#95926,#95927,#95928,#95929,
#95930,#95931,#95932,#95933,#95934,#95935,#95936,#95937,#95938,#95939,#95940,
#95941,#95942,#95943,#95944,#95945,#95946,#95947,#95948,#95949,#95950,#95951,
#95952,#95953,#95954,#95955,#95956,#95957,#95958,#95959,#95960,#95961,#95962,
#95963,#95964,#95965,#95966,#95967,#95968,#95969,#95970,#95971,#95972,#95973,
#95974,#95975,#95976,#95977,#95978,#95979,#95980,#95981,#95982,#95983,#95984,
#95985,#95986,#95987,#95988,#95989,#95990,#95991,#95992,#95993,#95994,#95995,
#95996,#95997,#95998,#95999,#96000,#96001,#96002,#96003,#96004,#96005,#96006,
#96007,#96008,#96009,#96010,#96011,#96012,#96013,#96014,#96015,#96016,#96017,
#96018,#96019,#96020,#96021,#96022,#96023,#96024,#96025,#96026,#96027,#96028,
#96029,#96030,#96031,#96032,#96033,#96034,#96035,#96036,#96037,#96038,#96039),
 .UNSPECIFIED.,.F.,.F.,(4,3,3,3,3,3,3,3,3,3,3,3,3,3,3,3,3,3,3,3,3,3,3,3,
3,3,3,3,3,3,3,3,3,3,3,3,3,3,3,3,3,3,3,3,3,3,3,3,3,3,3,3,3,3,3,3,3,3,3,3,
4),(70.4243747954073,70.5325790413758,70.6410991164241,70.7497863837822,
70.8587740112799,70.9173879472931,71.020782684341,71.124023966456,71.2271439318483,
71.3301985000572,71.4332217084149,71.5362475510874,71.6393803178655,71.7425694092753,
71.8459414026569,71.9162243972549,72.0196191343028,72.1228604164178,72.22598038181,
72.3290349500189,72.4320581583766,72.5350840010491,72.6382167678271,72.7414058592369,
72.8447778526185,72.9150608472168,73.0184555842648,73.1216968663798,73.2248168317721,
73.3278713999811,73.4308946083389,73.5339204510115,73.6370532177896,73.7402423091994,
73.8436143025811,73.9138972971787,74.0172920342266,74.1205333163416,74.2236532817339,
74.3267078499428,74.4297310583005,74.532756900973,74.6358896677511,74.7390787591609,
74.8424507525425,74.9127337471406,75.0161284841885,75.1193697663035,75.2224897316958,
75.3255442999047,75.4285675082624,75.5315933509349,75.6347261177129,75.7379152091227,
75.8412872025043,75.9115701971024,76.0134810050448,76.1152211478866,76.2168630906396,
76.3184433457412,76.3573194351122),.UNSPECIFIED.);
#955=B_SPLINE_CURVE_WITH_KNOTS('',3,(#96041,#96042,#96043,#96044,#96045,
#96046,#96047,#96048,#96049,#96050,#96051,#96052,#96053,#96054,#96055,#96056,
#96057,#96058,#96059,#96060,#96061,#96062,#96063,#96064,#96065,#96066,#96067,
#96068,#96069,#96070,#96071,#96072,#96073,#96074,#96075,#96076,#96077,#96078,
#96079,#96080,#96081,#96082,#96083,#96084,#96085,#96086,#96087,#96088,#96089,
#96090,#96091,#96092,#96093,#96094,#96095,#96096,#96097,#96098,#96099,#96100,
#96101,#96102,#96103,#96104,#96105,#96106,#96107,#96108,#96109,#96110,#96111,
#96112,#96113,#96114,#96115,#96116,#96117,#96118,#96119,#96120,#96121,#96122,
#96123,#96124,#96125,#96126,#96127,#96128,#96129,#96130,#96131,#96132,#96133,
#96134,#96135,#96136,#96137,#96138,#96139,#96140,#96141,#96142,#96143,#96144,
#96145,#96146,#96147,#96148,#96149,#96150,#96151,#96152,#96153,#96154,#96155,
#96156,#96157,#96158,#96159,#96160,#96161,#96162,#96163,#96164,#96165,#96166,
#96167,#96168,#96169,#96170,#96171,#96172,#96173,#96174,#96175,#96176,#96177,
#96178,#96179,#96180,#96181,#96182,#96183,#96184,#96185,#96186,#96187,#96188,
#96189,#96190,#96191,#96192,#96193,#96194,#96195,#96196,#96197,#96198,#96199,
#96200,#96201,#96202,#96203,#96204,#96205,#96206,#96207,#96208,#96209,#96210,
#96211,#96212,#96213,#96214,#96215,#96216,#96217,#96218,#96219,#96220,#96221,
#96222,#96223,#96224,#96225,#96226,#96227,#96228,#96229,#96230,#96231,#96232,
#96233,#96234,#96235,#96236,#96237,#96238,#96239,#96240,#96241,#96242,#96243,
#96244,#96245,#96246,#96247,#96248,#96249,#96250,#96251,#96252,#96253,#96254,
#96255,#96256),.UNSPECIFIED.,.F.,.F.,(4,2,2,2,2,2,2,2,2,2,2,2,2,2,2,2,2,
2,2,2,2,2,2,2,2,2,2,2,2,2,2,2,2,2,2,2,2,2,2,2,2,2,2,2,2,2,2,2,2,2,2,2,2,
2,2,2,2,2,2,2,2,2,2,2,2,2,2,2,2,2,2,2,2,2,2,2,2,2,2,2,2,2,2,2,2,2,2,2,2,
2,2,2,2,2,2,2,2,2,2,2,2,2,2,2,2,2,2,4),(-1.2596844006188,-1.23134348037588,
-1.22421236259465,-1.22130613130083,-1.21950569759933,-1.21754974270934,
-1.21487486052355,-1.20864136503829,-1.18159487613752,-1.1408667142172,
-1.11820860300803,-1.11535572922852,-1.113978945752,-1.11290509428865,-1.11166906535728,
-1.10949046530672,-1.09968793344074,-1.05077788864876,-1.01565733816867,
-1.01136168513588,-1.00882016943981,-1.0068792421472,-1.00480566806348,
-1.00155659103308,-0.991244539071412,-0.974681254939301,-0.941818681875961,
-0.928010773206015,-0.921314614232874,-0.9058651546604,-0.903497177917563,
-0.902089578195109,-0.901009419652921,-0.899805980301815,-0.897774221754095,
-0.889884499261976,-0.875168680537836,-0.846104322809252,-0.803698148398392,
-0.799404688837317,-0.796863865991712,-0.794923119346368,-0.792849400288268,
-0.789599390204754,-0.779278421619722,-0.762695147200479,-0.729816837435685,
-0.714514243732839,-0.709793809716609,-0.693941568323441,-0.691328755589958,
-0.689982898603794,-0.688911654783336,-0.687653737966812,-0.685374427280066,
-0.673948898758839,-0.647572543021168,-0.595122289837009,-0.58818879571284,
-0.585315752578351,-0.583521646009301,-0.581561193696602,-0.578859464446917,
-0.572467091901335,-0.526045725816737,-0.484947989958884,-0.480263111145685,
-0.478527326049579,-0.477502874716319,-0.476409871084484,-0.474895752896941,
-0.471290907393799,-0.432951749802275,-0.383317252134719,-0.376221628624632,
-0.373321716259422,-0.3715227255573,-0.36956638171457,-0.366887436208136,
-0.360806489500858,-0.352445554174214,-0.301550833652597,-0.270313243081288,
-0.267401275414166,-0.266013098530355,-0.264938282934619,-0.263710018326432,
-0.261566050213463,-0.25241497615479,-0.203666462142847,-0.167704290970596,
-0.162982357085103,-0.160559558854881,-0.158640677651432,-0.156487804187351,
-0.154258049263272,-0.146612099020315,-0.121083046625023,-0.100337619187811,
-0.0610229402291344,-0.0562870054891005,-0.0545435822959715,-0.0535177065254517,
-0.0524257939855512,-0.0509174411977632,-0.0492296227910852,-0.0462824128073364,
-0.000629120865108411),.UNSPECIFIED.);
#956=B_SPLINE_CURVE_WITH_KNOTS('',3,(#96257,#96258,#96259,#96260,#96261,
#96262,#96263,#96264,#96265,#96266,#96267,#96268,#96269),.UNSPECIFIED.,
 .F.,.F.,(4,3,3,3,4),(-66.6728921052185,-66.5709585796817,-66.4690950147616,
-66.3672509448711,-66.3228587574741),.UNSPECIFIED.);
#957=B_SPLINE_CURVE_WITH_KNOTS('',3,(#96274,#96275,#96276,#96277,#96278,
#96279,#96280,#96281,#96282,#96283,#96284,#96285,#96286,#96287,#96288,#96289,
#96290,#96291,#96292,#96293,#96294,#96295,#96296,#96297,#96298,#96299,#96300,
#96301,#96302,#96303,#96304,#96305,#96306,#96307,#96308,#96309,#96310,#96311,
#96312,#96313,#96314,#96315,#96316,#96317,#96318,#96319,#96320,#96321,#96322,
#96323,#96324,#96325,#96326,#96327,#96328,#96329,#96330,#96331,#96332,#96333,
#96334,#96335,#96336,#96337,#96338,#96339,#96340,#96341,#96342,#96343,#96344,
#96345,#96346,#96347,#96348,#96349,#96350,#96351,#96352,#96353,#96354,#96355,
#96356,#96357,#96358,#96359,#96360,#96361,#96362,#96363,#96364,#96365,#96366,
#96367,#96368,#96369,#96370,#96371,#96372,#96373,#96374,#96375,#96376,#96377,
#96378,#96379,#96380,#96381,#96382,#96383,#96384,#96385,#96386,#96387,#96388,
#96389,#96390,#96391,#96392,#96393,#96394,#96395,#96396,#96397,#96398,#96399,
#96400,#96401,#96402,#96403,#96404,#96405,#96406,#96407,#96408,#96409,#96410,
#96411,#96412,#96413,#96414,#96415,#96416,#96417,#96418,#96419,#96420,#96421,
#96422,#96423,#96424,#96425,#96426,#96427,#96428,#96429,#96430,#96431,#96432,
#96433,#96434,#96435,#96436,#96437,#96438,#96439,#96440,#96441,#96442,#96443,
#96444,#96445,#96446,#96447,#96448,#96449,#96450,#96451,#96452,#96453,#96454,
#96455,#96456,#96457,#96458,#96459,#96460,#96461,#96462,#96463,#96464,#96465,
#96466,#96467,#96468,#96469,#96470,#96471,#96472,#96473,#96474,#96475,#96476,
#96477,#96478,#96479,#96480,#96481,#96482,#96483,#96484,#96485,#96486,#96487,
#96488,#96489,#96490,#96491,#96492,#96493,#96494,#96495,#96496,#96497,#96498,
#96499,#96500,#96501,#96502,#96503,#96504,#96505,#96506,#96507),
 .UNSPECIFIED.,.F.,.F.,(4,2,2,2,2,2,2,2,2,2,2,2,2,2,2,2,2,2,2,2,2,2,2,2,
2,2,2,2,2,2,2,2,2,2,2,2,2,2,2,2,2,2,2,2,2,2,2,2,2,2,2,2,2,2,2,2,2,2,2,2,
2,2,2,2,2,2,2,2,2,2,2,2,2,2,2,2,2,2,2,2,2,2,2,2,2,2,2,2,2,2,2,2,2,2,2,2,
2,2,2,2,2,2,2,2,2,2,2,2,2,2,2,2,2,2,2,2,4),(-1.40849181731129,-1.39534413326025,
-1.3839435202864,-1.38166545110763,-1.38040770692253,-1.37933630327807,
-1.37798984927505,-1.37537471759749,-1.35945486214163,-1.3549530583211,
-1.33439091809116,-1.28603918699819,-1.27889054538664,-1.27598145261827,
-1.27418054699355,-1.27222510615025,-1.26955277515819,-1.26333365156747,
-1.2364027102941,-1.19587931431824,-1.17288882351002,-1.17003359567039,
-1.16865638586816,-1.16758253561546,-1.16634688497363,-1.16416985389905,
-1.15438934827788,-1.10546327810892,-1.07033832050305,-1.06604277856625,
-1.06350135239863,-1.0615605071805,-1.05948703406433,-1.05623814297163,
-1.04592691484572,-1.0293651759419,-0.996504733403481,-0.982762502489621,
-0.975913723538908,-0.975603980087717,-0.970099890012402,-0.960024116431277,
-0.957940683957954,-0.956603663469429,-0.955532937883248,-0.954268012591245,
-0.951956331220263,-0.939942367959669,-0.888190497283394,-0.858195618158027,
-0.853997984617839,-0.851485201816563,-0.849549119583362,-0.847463926274746,
-0.844161049461407,-0.833367529931291,-0.815723542794052,-0.765299615137646,
-0.764148951014091,-0.74855873040497,-0.745956883128004,-0.744613434252925,
-0.743542392477956,-0.742282718735769,-0.739995122329155,-0.728420923557461,
-0.701447117636352,-0.649842413473516,-0.642853031033282,-0.639970849521632,
-0.638175142299623,-0.636216220969492,-0.633522580024731,-0.627177323458069,
-0.599208688097817,-0.552613532096975,-0.536598391082022,-0.53397849141888,
-0.532631170900919,-0.531559912942187,-0.530303313659875,-0.52802978493932,
-0.516703247675675,-0.490716619276593,-0.437717077773332,-0.430825134330234,
-0.427959068462517,-0.426166334194717,-0.424204983883288,-0.421497624982962,
-0.415071182868322,-0.38642543851006,-0.335154364051163,-0.324142926650919,
-0.321999109401333,-0.320643665246783,-0.31957185619643,-0.318321414941718,
-0.316076127258167,-0.305228616952376,-0.281072259060738,-0.225373554692153,
-0.218721542979501,-0.215951841005866,-0.21400628797182,-0.212061424853581,
-0.210091687480759,-0.204924731766838,-0.160520234482066,-0.115647463093391,
-0.110925811268191,-0.109184560990818,-0.108159115366993,-0.1070669426203,
-0.105557060148865,-0.101976495484075,-0.0749220714811919),
 .UNSPECIFIED.);
#958=B_SPLINE_CURVE_WITH_KNOTS('',3,(#96509,#96510,#96511,#96512,#96513,
#96514,#96515,#96516,#96517,#96518,#96519,#96520,#96521,#96522,#96523,#96524,
#96525,#96526,#96527,#96528,#96529,#96530,#96531,#96532,#96533,#96534,#96535,
#96536,#96537,#96538,#96539,#96540,#96541,#96542,#96543,#96544,#96545,#96546,
#96547,#96548,#96549,#96550,#96551,#96552,#96553,#96554,#96555,#96556,#96557,
#96558,#96559,#96560,#96561,#96562,#96563,#96564,#96565,#96566,#96567,#96568,
#96569,#96570,#96571,#96572,#96573,#96574,#96575,#96576,#96577,#96578,#96579,
#96580,#96581,#96582,#96583,#96584,#96585,#96586,#96587,#96588,#96589,#96590,
#96591,#96592,#96593,#96594,#96595,#96596,#96597,#96598,#96599,#96600,#96601,
#96602,#96603,#96604,#96605,#96606,#96607,#96608,#96609,#96610,#96611,#96612,
#96613,#96614,#96615,#96616,#96617,#96618,#96619,#96620,#96621,#96622,#96623,
#96624,#96625,#96626,#96627,#96628,#96629,#96630,#96631,#96632,#96633,#96634,
#96635,#96636,#96637,#96638,#96639,#96640,#96641,#96642,#96643,#96644,#96645,
#96646,#96647,#96648,#96649,#96650,#96651,#96652,#96653,#96654,#96655,#96656,
#96657,#96658,#96659,#96660,#96661,#96662,#96663,#96664,#96665,#96666,#96667,
#96668,#96669,#96670,#96671,#96672,#96673,#96674,#96675,#96676,#96677,#96678,
#96679,#96680,#96681,#96682,#96683,#96684,#96685,#96686),.UNSPECIFIED.,
 .F.,.F.,(4,3,3,3,3,3,3,3,3,3,3,3,3,3,3,3,3,3,3,3,3,3,3,3,3,3,3,3,3,3,3,
3,3,3,3,3,3,3,3,3,3,3,3,3,3,3,3,3,3,3,3,3,3,3,3,3,3,3,3,4),(-66.3228587574741,
-66.2209269063509,-66.1189508258224,-66.0167874103627,-65.9232056974837,
-65.8198109604357,-65.7165696783208,-65.6134497129284,-65.5103951447194,
-65.4073719363617,-65.304346093689,-65.201213326911,-65.0980242355011,-64.9946522421195,
-64.9243692475218,-64.8209745104739,-64.7177332283588,-64.6146132629666,
-64.5115586947576,-64.4085354863999,-64.3055096437275,-64.2023768769495,
-64.0991877855397,-63.9958157921581,-63.9255327975599,-63.822138060512,
-63.718896778397,-63.6157768130047,-63.5127222447958,-63.4096990364379,
-63.3066731937653,-63.2035404269872,-63.1003513355775,-62.9969793421958,
-62.9266963475981,-62.8233016105502,-62.7200603284354,-62.6169403630432,
-62.5138857948343,-62.4108625864766,-62.3078367438041,-62.2047039770261,
-62.1015148856163,-61.9981428922347,-61.9278598976362,-61.8244651605881,
-61.7212238784729,-61.6181039130806,-61.5150493448717,-61.412026136514,
-61.3090002938412,-61.2058675270631,-61.1026784356533,-60.9993064422715,
-60.9290234476743,-60.8220651862385,-60.7139755891886,-60.6074364851719,
-60.4985716416054,-60.3897067980389),.UNSPECIFIED.);
#959=B_SPLINE_CURVE_WITH_KNOTS('',3,(#96687,#96688,#96689,#96690),
 .UNSPECIFIED.,.F.,.F.,(4,4),(-60.3897037700523,-60.0402339956293),
 .UNSPECIFIED.);
#960=B_SPLINE_CURVE_WITH_KNOTS('',3,(#96696,#96697,#96698,#96699,#96700,
#96701),.UNSPECIFIED.,.F.,.F.,(4,2,4),(-0.075038806717288,-0.0529910440511674,
-0.000629600917318996),.UNSPECIFIED.);
#961=B_SPLINE_CURVE_WITH_KNOTS('',3,(#96702,#96703,#96704,#96705,#96706,
#96707,#96708,#96709,#96710,#96711,#96712,#96713,#96714,#96715,#96716,#96717,
#96718,#96719,#96720,#96721,#96722,#96723,#96724,#96725,#96726,#96727,#96728,
#96729,#96730,#96731,#96732,#96733,#96734,#96735,#96736,#96737,#96738,#96739,
#96740,#96741,#96742,#96743,#96744,#96745,#96746,#96747,#96748,#96749,#96750,
#96751,#96752,#96753,#96754,#96755,#96756,#96757,#96758,#96759,#96760,#96761,
#96762,#96763,#96764,#96765,#96766,#96767,#96768,#96769,#96770,#96771,#96772,
#96773,#96774,#96775,#96776,#96777,#96778,#96779,#96780,#96781,#96782,#96783,
#96784,#96785,#96786,#96787,#96788,#96789,#96790,#96791,#96792,#96793,#96794,
#96795,#96796,#96797,#96798,#96799,#96800,#96801,#96802,#96803,#96804,#96805,
#96806,#96807,#96808,#96809,#96810,#96811,#96812,#96813,#96814,#96815,#96816,
#96817,#96818,#96819,#96820,#96821,#96822,#96823,#96824,#96825,#96826,#96827,
#96828,#96829,#96830,#96831,#96832,#96833,#96834,#96835,#96836,#96837,#96838,
#96839,#96840,#96841,#96842,#96843,#96844,#96845,#96846,#96847,#96848,#96849,
#96850,#96851,#96852,#96853,#96854,#96855,#96856,#96857,#96858,#96859,#96860,
#96861,#96862,#96863,#96864,#96865,#96866,#96867,#96868,#96869,#96870,#96871,
#96872,#96873,#96874,#96875,#96876,#96877,#96878,#96879,#96880,#96881,#96882,
#96883,#96884,#96885,#96886,#96887,#96888,#96889,#96890,#96891,#96892,#96893,
#96894,#96895,#96896,#96897,#96898,#96899,#96900,#96901,#96902,#96903,#96904,
#96905,#96906,#96907,#96908,#96909,#96910,#96911,#96912,#96913,#96914,#96915,
#96916,#96917,#96918,#96919,#96920,#96921,#96922,#96923,#96924,#96925,#96926,
#96927,#96928,#96929,#96930,#96931,#96932,#96933,#96934,#96935,#96936,#96937,
#96938,#96939,#96940,#96941,#96942,#96943,#96944,#96945,#96946,#96947,#96948,
#96949,#96950,#96951),.UNSPECIFIED.,.F.,.F.,(4,2,2,2,2,2,2,2,2,2,2,2,2,
2,2,2,2,2,2,2,2,2,2,2,2,2,2,2,2,2,2,2,2,2,2,2,2,2,2,2,2,2,2,2,2,2,2,2,2,
2,2,2,2,2,2,2,2,2,2,2,2,2,2,2,2,2,2,2,2,2,2,2,2,2,2,2,2,2,2,2,2,2,2,2,2,
2,2,2,2,2,2,2,2,2,2,2,2,2,2,2,2,2,2,2,2,2,2,2,2,2,2,2,2,2,2,2,2,2,2,2,2,
2,2,2,4),(-2.66785867798683,-2.65980139307743,-2.65544393569796,-2.65403085994829,
-2.65296354475938,-2.65193327423883,-2.65075329188821,-2.64882796290568,
-2.64276206648497,-2.64147998045497,-2.63367912055449,-2.58042654028585,
-2.56271330019522,-2.55188924146064,-2.54858214767669,-2.54649548013368,
-2.54455884793956,-2.54204651216505,-2.53785220327919,-2.50806282802426,
-2.46716795538772,-2.45178619053623,-2.44638418086373,-2.44378952291186,
-2.44168554628189,-2.44047341238879,-2.44047028729506,-2.44046714336841,
-2.44046398041027,-2.4404607982075,-2.4404575964406,-2.44045437500728,-2.44045113396158,
-2.44044787324233,-2.44044459246466,-2.44044129128748,-2.44043796991524,
-2.44043464134687,-2.4404312983739,-2.44042793429552,-2.44042454900457,
-2.44042113116944,-2.43939351501871,-2.43801460546967,-2.43515022177071,
-2.39947437974768,-2.36660902743931,-2.34389542618647,-2.33822104087803,
-2.33564591823926,-2.3337068396424,-2.33188121406708,-2.32934345565815,
-2.3227290257416,-2.26665380577393,-2.24276557413512,-2.23198914584977,
-2.22974796872575,-2.22849831188082,-2.22742625047205,-2.22606929292911,
-2.22392083108199,-2.21283818601615,-2.16155989913174,-2.13294209920106,
-2.126519122556,-2.12381216793253,-2.12185072945635,-2.12005765621856,-2.11719047436762,
-2.11029284835065,-2.05738495188888,-2.0313576970674,-2.02001968913433,
-2.01774536097607,-2.01648850666873,-2.01541714820455,-2.01406984381859,
-2.01145039637796,-1.99544564797781,-1.98996784299213,-1.97552292411418,
-1.94263073634456,-1.92606484837104,-1.91575271974157,-1.91250367583362,
-1.91043014304709,-1.90848926910961,-1.90594784570508,-1.90165243100518,
-1.86652427307357,-1.81757324781445,-1.80785368827791,-1.80568087658229,
-1.80444616302768,-1.80337219775383,-1.8019936149713,-1.79913133340986,
-1.76311285885758,-1.7303606436664,-1.70782644079248,-1.70217602943133,
-1.69960515224254,-1.69766657115448,-1.69583943065096,-1.69329638422362,
-1.68664930700714,-1.63088184758667,-1.59797879193682,-1.59443218587794,
-1.59292787761089,-1.59183643955113,-1.59080905051046,-1.58905884570364,
-1.58428012273461,-1.5471131285102,-1.49683942494867,-1.49043745040415,
-1.48773388174164,-1.48577290593268,-1.48397888354758,-1.48110719266454,
-1.47418323057818,-1.4216167136691,-1.40849181731129),.UNSPECIFIED.);
#962=B_SPLINE_CURVE_WITH_KNOTS('',3,(#96953,#96954,#96955,#96956,#96957,
#96958,#96959,#96960,#96961,#96962),.UNSPECIFIED.,.F.,.F.,(4,1,1,1,1,1,
1,4),(-60.0402339956293,-59.9301869977125,-58.9313505477506,-57.9325140977887,
-56.9336776478268,-55.934841197865,-54.9360047479031,-54.1065275196936),
 .UNSPECIFIED.);
#963=B_SPLINE_CURVE_WITH_KNOTS('',3,(#96963,#96964,#96965,#96966,#96967,
#96968,#96969,#96970,#96971,#96972,#96973,#96974,#96975,#96976,#96977,#96978,
#96979,#96980,#96981,#96982,#96983,#96984),.UNSPECIFIED.,.F.,.F.,(4,2,2,
2,2,2,2,2,2,2,4),(-2.66748285763103,-2.64324926503545,-2.63611726584707,
-2.63432648362479,-2.63311152542526,-2.63210237517397,-2.63102767404166,
-2.62964130759543,-2.62673900317765,-2.59968632690069,-2.59337489789675),
 .UNSPECIFIED.);
#964=B_SPLINE_CURVE_WITH_KNOTS('',3,(#96989,#96990,#96991,#96992,#96993,
#96994,#96995,#96996,#96997,#96998,#96999,#97000,#97001,#97002,#97003,#97004,
#97005,#97006,#97007,#97008,#97009,#97010,#97011,#97012,#97013,#97014,#97015,
#97016,#97017,#97018,#97019,#97020,#97021,#97022,#97023,#97024,#97025,#97026,
#97027,#97028,#97029,#97030,#97031,#97032,#97033,#97034,#97035,#97036,#97037,
#97038,#97039,#97040,#97041,#97042,#97043,#97044,#97045,#97046,#97047,#97048,
#97049,#97050,#97051,#97052,#97053,#97054,#97055,#97056,#97057,#97058,#97059,
#97060,#97061,#97062,#97063,#97064,#97065,#97066,#97067,#97068,#97069,#97070,
#97071,#97072,#97073,#97074,#97075,#97076,#97077,#97078,#97079,#97080,#97081,
#97082,#97083,#97084,#97085,#97086,#97087,#97088,#97089,#97090,#97091,#97092,
#97093,#97094,#97095,#97096,#97097,#97098,#97099,#97100,#97101,#97102,#97103,
#97104,#97105,#97106,#97107,#97108,#97109,#97110,#97111,#97112,#97113,#97114,
#97115,#97116,#97117,#97118,#97119,#97120,#97121,#97122,#97123,#97124,#97125,
#97126,#97127,#97128,#97129,#97130,#97131,#97132,#97133,#97134,#97135,#97136,
#97137,#97138,#97139,#97140,#97141,#97142,#97143,#97144,#97145,#97146,#97147,
#97148,#97149,#97150,#97151,#97152,#97153,#97154,#97155,#97156,#97157,#97158,
#97159,#97160,#97161,#97162,#97163,#97164,#97165,#97166,#97167,#97168,#97169,
#97170,#97171,#97172,#97173,#97174,#97175,#97176,#97177,#97178,#97179,#97180,
#97181,#97182,#97183,#97184,#97185,#97186,#97187,#97188,#97189,#97190,#97191,
#97192,#97193,#97194,#97195,#97196,#97197,#97198,#97199,#97200,#97201,#97202,
#97203,#97204,#97205,#97206,#97207,#97208,#97209,#97210,#97211,#97212,#97213,
#97214,#97215,#97216,#97217,#97218,#97219,#97220,#97221,#97222,#97223,#97224,
#97225,#97226,#97227,#97228,#97229,#97230),.UNSPECIFIED.,.F.,.F.,(4,2,2,
2,2,2,2,2,2,2,2,2,2,2,2,2,2,2,2,2,2,2,2,2,2,2,2,2,2,2,2,2,2,2,2,2,2,2,2,
2,2,2,2,2,2,2,2,2,2,2,2,2,2,2,2,2,2,2,2,2,2,2,2,2,2,2,2,2,2,2,2,2,2,2,2,
2,2,2,2,2,2,2,2,2,2,2,2,2,2,2,2,2,2,2,2,2,2,2,2,2,2,2,2,2,2,2,2,2,2,2,2,
2,2,2,2,2,2,2,2,2,4),(-1.40848019473541,-1.38239422892346,-1.36905396071534,
-1.36549889522737,-1.36335772755904,-1.36143643340249,-1.35899308762589,
-1.35511850832949,-1.33404421585164,-1.27622795910977,-1.26126705211177,
-1.25891899021377,-1.25751716473004,-1.25643775943186,-1.25523107519433,
-1.25318491262186,-1.24512732575371,-1.22994776179928,-1.19005056034978,
-1.15900595251883,-1.15478430885474,-1.15226431199618,-1.15032685172039,
-1.14824428466472,-1.14495430607332,-1.13428040366213,-1.11690862295099,
-1.06820376947828,-1.0616881803853,-1.04906566855534,-1.04682990993342,
-1.0454464620129,-1.04437201164759,-1.04314046352743,-1.04098203999855,
-1.03146950600333,-0.982315198169504,-0.947118886371042,-0.942822455217987,
-0.940280786188271,-0.938339918592029,-0.936266579679289,-0.933018228955314,
-0.922711497671774,-0.906159626264462,-0.873307589385927,-0.86038887438955,
-0.837685948899323,-0.834832345499673,-0.833455550912708,-0.832381851188896,
-0.831146178093623,-0.828968639073795,-0.819178084796704,-0.770267216652909,
-0.735149493413028,-0.730854498440486,-0.728313383490019,-0.726372768806855,
-0.724299535060604,-0.721051004586173,-0.710740799187361,-0.694180587140001,
-0.661323663265587,-0.647548901024741,-0.640781714200325,-0.639209642602496,
-0.625256611023007,-0.622954753772721,-0.621566632822581,-0.620489225944818,
-0.619275182724371,-0.61719517154778,-0.608722294385308,-0.59235999035848,
-0.550186061678572,-0.522931311232696,-0.51880379994111,-0.516311646422943,
-0.514378814354156,-0.512284527687986,-0.508940075826187,-0.497761100931318,
-0.479229583265353,-0.434842373529562,-0.413730454697519,-0.410917775636129,
-0.409549153375782,-0.408476318783945,-0.407235382109819,-0.405033425329507,
-0.394874207177727,-0.373180133958159,-0.372020402648616,-0.313853998860858,
-0.307478907457946,-0.304980419143423,-0.303165297711273,-0.301220790141232,
-0.298609755306034,-0.292735714533123,-0.268516125991691,-0.227082755051121,
-0.201866987532232,-0.198983098684127,-0.197600547825018,-0.19657105381372,
-0.19538021786063,-0.193408432882404,-0.190985475666953,-0.18607475251318,
-0.172714987700871,-0.15252651232384,-0.102928705546204,-0.0958339839794316,
-0.0929345388287951,-0.0911358677574391,-0.0891798950949667,-0.0865015004779375,
-0.0802438387687248,-0.075038806717288),.UNSPECIFIED.);
#965=B_SPLINE_CURVE_WITH_KNOTS('',3,(#97231,#97232,#97233,#97234,#97235,
#97236,#97237,#97238,#97239,#97240,#97241,#97242,#97243,#97244,#97245,#97246,
#97247,#97248,#97249,#97250,#97251,#97252,#97253,#97254,#97255,#97256,#97257,
#97258,#97259,#97260,#97261,#97262,#97263,#97264,#97265,#97266,#97267,#97268,
#97269,#97270,#97271,#97272,#97273,#97274,#97275,#97276,#97277,#97278,#97279,
#97280,#97281,#97282,#97283,#97284,#97285,#97286,#97287,#97288,#97289,#97290,
#97291,#97292,#97293,#97294,#97295,#97296,#97297,#97298,#97299,#97300,#97301,
#97302,#97303,#97304,#97305,#97306,#97307,#97308,#97309,#97310,#97311,#97312,
#97313,#97314,#97315,#97316,#97317,#97318,#97319,#97320,#97321,#97322,#97323,
#97324,#97325,#97326,#97327,#97328,#97329,#97330,#97331,#97332,#97333,#97334,
#97335,#97336,#97337,#97338,#97339,#97340,#97341,#97342,#97343,#97344,#97345,
#97346,#97347,#97348,#97349,#97350,#97351,#97352,#97353,#97354,#97355,#97356,
#97357,#97358,#97359,#97360,#97361,#97362,#97363,#97364,#97365,#97366,#97367,
#97368,#97369,#97370,#97371,#97372,#97373,#97374,#97375,#97376,#97377,#97378,
#97379,#97380,#97381,#97382,#97383,#97384,#97385,#97386,#97387,#97388,#97389,
#97390,#97391,#97392,#97393,#97394,#97395,#97396,#97397,#97398,#97399,#97400,
#97401,#97402,#97403,#97404,#97405,#97406,#97407,#97408,#97409,#97410,#97411,
#97412,#97413,#97414,#97415,#97416,#97417,#97418,#97419,#97420,#97421,#97422,
#97423,#97424,#97425,#97426,#97427,#97428,#97429,#97430,#97431,#97432,#97433,
#97434,#97435,#97436,#97437,#97438,#97439,#97440,#97441,#97442,#97443,#97444,
#97445,#97446,#97447,#97448,#97449,#97450,#97451,#97452,#97453,#97454,#97455,
#97456,#97457,#97458,#97459,#97460,#97461,#97462),.UNSPECIFIED.,.F.,.F.,
(4,2,2,2,2,2,2,2,2,2,2,2,2,2,2,2,2,2,2,2,2,2,2,2,2,2,2,2,2,2,2,2,2,2,2,
2,2,2,2,2,2,2,2,2,2,2,2,2,2,2,2,2,2,2,2,2,2,2,2,2,2,2,2,2,2,2,2,2,2,2,2,
2,2,2,2,2,2,2,2,2,2,2,2,2,2,2,2,2,2,2,2,2,2,2,2,2,2,2,2,2,2,2,2,2,2,2,2,
2,2,2,2,2,2,2,2,4),(-2.59337489789675,-2.58561238519003,-2.5736012351672,
-2.54190221097263,-2.53146041821309,-2.52819650651114,-2.5261196695812,
-2.52418002920341,-2.52164644052308,-2.51737815087784,-2.47198908962061,
-2.43802611821553,-2.42427914629956,-2.42171890202092,-2.42039483697899,
-2.41932314271042,-2.41806909731193,-2.41586843293411,-2.40685723000472,
-2.3539464386988,-2.32470989911176,-2.3182134621207,-2.31549409417234,-2.31353034358247,
-2.31173973576514,-2.30888641642316,-2.30207328760224,-2.24810944652342,
-2.2228088075181,-2.21165735957861,-2.20939377507873,-2.20813922927116,
-2.20706762767805,-2.20571719678519,-2.20308334374152,-2.18672590873896,
-2.1365525419151,-2.11849488894645,-2.10752136554714,-2.10419864685843,
-2.10210896322935,-2.10017422282583,-2.0976709568711,-2.09350624250701,
-2.06484193251605,-2.02312196497596,-2.0075113351921,-1.99929969366833,
-1.99724077921504,-1.9960313206454,-1.99495270339727,-1.99355614494871,
-1.99122585914714,-1.97668180279041,-1.97434015171541,-1.92392035721741,
-1.90628580118414,-1.89549740629227,-1.89219500059953,-1.89010985851512,
-1.88817365467598,-1.885660475484,-1.88146168600695,-1.85141120350088,-1.79974569391282,
-1.78774105761309,-1.78542990109675,-1.78416508566437,-1.78309435054852,
-1.78175718392715,-1.77967326754144,-1.76959081022052,-1.76408866920562,
-1.75666075903552,-1.74315374735036,-1.7102720985274,-1.69371845410015,
-1.68341191728806,-1.68016355512271,-1.6780901978289,-1.67614930578707,
-1.67360759552205,-1.66931110610758,-1.63409411711189,-1.58484929870086,
-1.57547164839891,-1.57332286152462,-1.57209345272159,-1.57101869294232,
-1.56963197057584,-1.56738526024835,-1.55455239771529,-1.55238635613203,
-1.50510602602108,-1.47658192153856,-1.47016996644554,-1.46746478530359,
-1.46550358715487,-1.46371001402097,-1.4608404651189,-1.45392902539541,
-1.40119799850049,-1.37504370370648,-1.36367320927299,-1.3613969336009,
-1.36013961456057,-1.35906823067263,-1.35772136595842,-1.35510415844712,
-1.33914219057051,-1.33419819696957,-1.32855219827746,-1.2815931219422,
-1.28014709804074,-1.26110786927851,-1.25973005914825),.UNSPECIFIED.);
#966=B_SPLINE_CURVE_WITH_KNOTS('',3,(#97468,#97469,#97470,#97471,#97472,
#97473,#97474,#97475,#97476,#97477,#97478,#97479,#97480,#97481,#97482,#97483),
 .UNSPECIFIED.,.F.,.F.,(4,2,2,2,2,2,2,4),(-0.0747630397369221,-0.074125929836722,
-0.0730538955052031,-0.0718062276008534,-0.0695734668952728,-0.0589294385692646,
-0.0355200016789157,-0.000629543070150967),.UNSPECIFIED.);
#967=B_SPLINE_CURVE_WITH_KNOTS('',3,(#97484,#97485,#97486,#97487,#97488,
#97489,#97490,#97491,#97492,#97493,#97494,#97495,#97496,#97497,#97498,#97499,
#97500,#97501,#97502,#97503,#97504,#97505,#97506,#97507,#97508,#97509,#97510,
#97511,#97512,#97513,#97514,#97515,#97516,#97517,#97518,#97519,#97520,#97521,
#97522,#97523,#97524,#97525,#97526,#97527,#97528,#97529,#97530,#97531,#97532,
#97533,#97534,#97535,#97536,#97537,#97538,#97539,#97540,#97541,#97542,#97543,
#97544,#97545,#97546,#97547,#97548,#97549,#97550,#97551,#97552,#97553,#97554,
#97555,#97556,#97557,#97558,#97559,#97560,#97561,#97562,#97563,#97564,#97565,
#97566,#97567,#97568,#97569,#97570,#97571,#97572,#97573,#97574,#97575,#97576,
#97577,#97578,#97579,#97580,#97581,#97582,#97583,#97584,#97585,#97586,#97587,
#97588,#97589,#97590,#97591,#97592,#97593,#97594,#97595,#97596,#97597,#97598,
#97599,#97600,#97601,#97602,#97603,#97604,#97605,#97606,#97607,#97608,#97609,
#97610,#97611,#97612,#97613,#97614,#97615,#97616,#97617,#97618,#97619,#97620,
#97621,#97622,#97623,#97624,#97625,#97626,#97627,#97628,#97629,#97630,#97631,
#97632,#97633,#97634,#97635,#97636,#97637,#97638,#97639,#97640,#97641,#97642,
#97643,#97644,#97645,#97646,#97647,#97648,#97649,#97650,#97651,#97652,#97653,
#97654,#97655,#97656,#97657,#97658,#97659,#97660,#97661,#97662,#97663,#97664,
#97665,#97666,#97667,#97668,#97669,#97670,#97671,#97672,#97673,#97674,#97675,
#97676,#97677,#97678,#97679,#97680,#97681,#97682,#97683,#97684,#97685,#97686,
#97687,#97688,#97689,#97690,#97691,#97692,#97693,#97694,#97695,#97696,#97697,
#97698,#97699,#97700,#97701,#97702,#97703,#97704,#97705,#97706,#97707),
 .UNSPECIFIED.,.F.,.F.,(4,2,2,2,2,2,2,2,2,2,2,2,2,2,2,2,2,2,2,2,2,2,2,2,
2,2,2,2,2,2,2,2,2,2,2,2,2,2,2,2,2,2,2,2,2,2,2,2,2,2,2,2,2,2,2,2,2,2,2,2,
2,2,2,2,2,2,2,2,2,2,2,2,2,2,2,2,2,2,2,2,2,2,2,2,2,2,2,2,2,2,2,2,2,2,2,2,
2,2,2,2,2,2,2,2,2,2,2,2,2,2,2,4),(-2.66783535108714,-2.64250906893,-2.63938208222713,
-2.63723600115051,-2.63543519243453,-2.63352124181565,-2.6311520769427,
-2.62751851804251,-2.61041314579988,-2.59822256861164,-2.5565501005403,
-2.54066441939936,-2.53235654636494,-2.53028999587732,-2.52907899257403,
-2.52800100808561,-2.52660787969764,-2.52428879783054,-2.51000006914887,
-2.50120107583317,-2.47962900749421,-2.44818170163269,-2.43607186156944,
-2.43058444851967,-2.42623476187509,-2.42393221098337,-2.4220195563318,
-2.41981678698706,-2.4160800392244,-2.40203629057023,-2.34395278460679,
-2.32851772707835,-2.32036856462133,-2.31831495680088,-2.3171067402988,
-2.31602794103389,-2.3146294660068,-2.31229243423733,-2.2975890856737,-2.25146107462409,
-2.22185180691862,-2.21531195362349,-2.21258551123426,-2.21062062485524,
-2.20883169361043,-2.20598689151067,-2.19922377643746,-2.14470006903296,
-2.11978692981944,-2.10873726059878,-2.10647984098072,-2.10522672175815,
-2.10415512154941,-2.10280313681509,-2.10016163887205,-2.08360356604286,
-2.03306548313488,-2.00887727263476,-2.0030074260505,-2.00039697573588,
-1.99845240207015,-1.99663686178176,-1.99413723572669,-1.98775622038017,
-1.92965504297113,-1.90706106013365,-1.89664309510086,-1.89442434029175,
-1.8931796447804,-1.89210714062645,-1.89074355824237,-1.88857313871593,
-1.87712455004244,-1.87307012438648,-1.8728248183821,-1.86595929124893,
-1.852225984038,-1.81934327750738,-1.80278750071601,-1.79248010429687,-1.78923172022595,
-1.78715840879499,-1.78521760172687,-1.78267606340333,-1.77838000061332,
-1.74318521068846,-1.69401409937404,-1.68455450257467,-1.68239993056173,
-1.68116927475662,-1.68009476271526,-1.67871012021756,-1.67581660956862,
-1.6497822965264,-1.61161487953928,-1.58258677680828,-1.5781911436166,-1.57586756012254,
-1.57395594501301,-1.57173181097133,-1.5679035370945,-1.55284212658676,
-1.50067345456839,-1.4818277802287,-1.47253189567416,-1.47038898712396,
-1.46916087139268,-1.4680858926064,-1.4666971069231,-1.46378247467635,-1.43373616217968,
-1.40848019473541),.UNSPECIFIED.);
#968=B_SPLINE_CURVE_WITH_KNOTS('',3,(#97709,#97710,#97711,#97712,#97713,
#97714,#97715,#97716,#97717,#97718,#97719,#97720,#97721,#97722,#97723,#97724,
#97725,#97726,#97727,#97728,#97729,#97730,#97731,#97732,#97733,#97734,#97735,
#97736,#97737,#97738,#97739,#97740,#97741,#97742,#97743,#97744,#97745,#97746,
#97747,#97748,#97749,#97750,#97751,#97752,#97753,#97754,#97755,#97756,#97757,
#97758,#97759,#97760,#97761,#97762,#97763,#97764,#97765,#97766,#97767,#97768,
#97769,#97770,#97771,#97772,#97773,#97774,#97775,#97776,#97777,#97778,#97779,
#97780,#97781,#97782,#97783,#97784,#97785,#97786,#97787,#97788,#97789,#97790,
#97791,#97792,#97793,#97794,#97795,#97796,#97797,#97798,#97799,#97800,#97801,
#97802,#97803,#97804,#97805,#97806,#97807,#97808,#97809,#97810,#97811,#97812,
#97813,#97814,#97815,#97816,#97817,#97818,#97819,#97820,#97821,#97822,#97823,
#97824,#97825,#97826,#97827,#97828,#97829,#97830,#97831,#97832,#97833,#97834,
#97835,#97836,#97837,#97838,#97839,#97840,#97841,#97842,#97843,#97844,#97845,
#97846,#97847,#97848,#97849,#97850,#97851,#97852,#97853,#97854,#97855,#97856,
#97857,#97858,#97859,#97860,#97861,#97862,#97863,#97864,#97865,#97866,#97867,
#97868,#97869,#97870,#97871,#97872,#97873,#97874,#97875,#97876,#97877,#97878,
#97879,#97880,#97881,#97882,#97883,#97884,#97885,#97886,#97887,#97888,#97889,
#97890,#97891,#97892,#97893,#97894,#97895,#97896,#97897,#97898,#97899,#97900,
#97901,#97902,#97903,#97904,#97905,#97906,#97907,#97908,#97909,#97910,#97911,
#97912,#97913,#97914,#97915,#97916,#97917,#97918,#97919,#97920,#97921,#97922,
#97923,#97924,#97925,#97926),.UNSPECIFIED.,.F.,.F.,(4,2,2,2,2,2,2,2,2,2,
2,2,2,2,2,2,2,2,2,2,2,2,2,2,2,2,2,2,2,2,2,2,2,2,2,2,2,2,2,2,2,2,2,2,2,2,
2,2,2,2,2,2,2,2,2,2,2,2,2,2,2,2,2,2,2,2,2,2,2,2,2,2,2,2,2,2,2,2,2,2,2,2,
2,2,2,2,2,2,2,2,2,2,2,2,2,2,2,2,2,2,2,2,2,2,2,2,2,2,4),(-1.25973005914825,
-1.25734673576451,-1.25493799364887,-1.25302024499271,-1.25085804788037,
-1.24720822119141,-1.23275560773671,-1.18236883734888,-1.15270137220804,
-1.14978688828851,-1.1483981269892,-1.1473231419446,-1.14609500024645,-1.14395198793024,
-1.13465505386342,-1.11580362506527,-1.07535049127943,-1.06307183334997,
-1.04849206650873,-1.04470610185088,-1.04249165398581,-1.04057937096035,
-1.03824369402508,-1.03379063115923,-1.0027547532014,-0.954777987487901,
-0.940188301453422,-0.937855920131238,-0.936458678044927,-0.935379884791108,
-0.934170633265356,-0.932112949431952,-0.923917837684583,-0.908352484961321,
-0.866771608499126,-0.854699776541554,-0.836944049735642,-0.833267517262526,
-0.830884743673292,-0.828969247295901,-0.82678973231593,-0.823061740997188,
-0.807614707829557,-0.756014456353178,-0.728679189755335,-0.725774778178223,
-0.724387941036871,-0.723313118750484,-0.722083677207734,-0.719934909918138,
-0.710558854482192,-0.661284061362405,-0.626051867018526,-0.621754867939458,
-0.619212998049116,-0.617272054867228,-0.615198710624219,-0.611950508975189,
-0.601645577007871,-0.58509785607852,-0.552248725360138,-0.539753922742267,
-0.516621401094841,-0.513763498712775,-0.512385837313556,-0.511312028791543,
-0.51007687077048,-0.507901770803435,-0.49814751764719,-0.449204429645168,
-0.414076923548904,-0.409780950983742,-0.407239516710465,-0.405298807344663,
-0.403225617073029,-0.399977456669936,-0.389670970747025,-0.373119152827878,
-0.340268659111501,-0.327240365109306,-0.318507978720654,-0.304211753872246,
-0.301892029381645,-0.300498637562593,-0.299420526714317,-0.298209479819172,
-0.296143057872224,-0.287838601264404,-0.271961271137324,-0.225895406465433,
-0.201639020674606,-0.1976237345401,-0.195164705357662,-0.193294628387892,
-0.19126654636763,-0.188075316889398,-0.184320141673537,-0.177183987718724,
-0.15961252712563,-0.109463964776951,-0.0924352898109446,-0.089776066101595,
-0.088420321839725,-0.087348495859116,-0.0860982883850014,-0.083854053618281,
-0.0730237950007372,-0.0489314110027095,-0.000629479462340787),
 .UNSPECIFIED.);
#969=B_SPLINE_CURVE_WITH_KNOTS('',3,(#97927,#97928,#97929,#97930,#97931,
#97932,#97933,#97934,#97935,#97936,#97937,#97938,#97939,#97940,#97941,#97942,
#97943,#97944,#97945,#97946,#97947,#97948),.UNSPECIFIED.,.F.,.F.,(4,2,2,
2,2,2,2,2,2,2,4),(-2.6678214478774,-2.66002753739846,-2.6547310404401,-2.65228763735666,
-2.65040576350708,-2.64856503657601,-2.64673861360468,-2.64419819355603,
-2.63900696606325,-2.62649661765704,-2.59340742691029),.UNSPECIFIED.);
#970=B_SPLINE_CURVE_WITH_KNOTS('',3,(#97953,#97954,#97955,#97956,#97957,
#97958,#97959,#97960,#97961,#97962,#97963,#97964,#97965,#97966,#97967,#97968,
#97969,#97970,#97971,#97972,#97973,#97974,#97975,#97976,#97977,#97978,#97979,
#97980,#97981,#97982,#97983,#97984,#97985,#97986,#97987,#97988,#97989,#97990,
#97991,#97992,#97993,#97994,#97995,#97996,#97997,#97998,#97999,#98000,#98001,
#98002,#98003,#98004,#98005,#98006,#98007,#98008,#98009,#98010,#98011,#98012,
#98013,#98014,#98015,#98016,#98017,#98018,#98019,#98020,#98021,#98022,#98023,
#98024,#98025,#98026,#98027,#98028,#98029,#98030,#98031,#98032,#98033,#98034,
#98035,#98036,#98037,#98038,#98039,#98040,#98041,#98042,#98043,#98044,#98045,
#98046,#98047,#98048,#98049,#98050,#98051,#98052,#98053,#98054,#98055,#98056,
#98057,#98058,#98059,#98060,#98061,#98062,#98063,#98064,#98065,#98066,#98067,
#98068,#98069,#98070,#98071,#98072,#98073,#98074,#98075,#98076,#98077,#98078,
#98079,#98080,#98081,#98082,#98083,#98084,#98085,#98086,#98087,#98088,#98089,
#98090,#98091,#98092,#98093,#98094,#98095,#98096,#98097,#98098,#98099,#98100,
#98101,#98102,#98103,#98104,#98105,#98106,#98107,#98108,#98109,#98110,#98111,
#98112,#98113,#98114,#98115,#98116,#98117,#98118,#98119,#98120,#98121,#98122,
#98123,#98124,#98125,#98126,#98127,#98128,#98129,#98130,#98131,#98132,#98133,
#98134,#98135,#98136,#98137,#98138,#98139,#98140,#98141,#98142,#98143,#98144,
#98145,#98146,#98147,#98148,#98149,#98150,#98151,#98152,#98153,#98154,#98155,
#98156,#98157,#98158,#98159,#98160,#98161,#98162,#98163,#98164,#98165,#98166,
#98167,#98168,#98169,#98170,#98171,#98172,#98173,#98174),.UNSPECIFIED.,
 .F.,.F.,(4,2,2,2,2,2,2,2,2,2,2,2,2,2,2,2,2,2,2,2,2,2,2,2,2,2,2,2,2,2,2,
2,2,2,2,2,2,2,2,2,2,2,2,2,2,2,2,2,2,2,2,2,2,2,2,2,2,2,2,2,2,2,2,2,2,2,2,
2,2,2,2,2,2,2,2,2,2,2,2,2,2,2,2,2,2,2,2,2,2,2,2,2,2,2,2,2,2,2,2,2,2,2,2,
2,2,2,2,2,2,2,4),(-1.40845787076926,-1.36760548623614,-1.35571294198462,
-1.35117785792175,-1.34786945228156,-1.3464069708187,-1.34532226889899,
-1.34413338184527,-1.34216743748543,-1.3357623369736,-1.33420643238553,
-1.31961991307284,-1.26057847745824,-1.24626880242789,-1.2425071213422,
-1.24029829200361,-1.23838564018709,-1.23604291757183,-1.23155599889841,
-1.19919435451072,-1.15901049115682,-1.15407864423868,-1.13812964660466,
-1.13551314136766,-1.13416643685508,-1.13309507396208,-1.13183766177518,
-1.12956090710595,-1.11818217252907,-1.09199256927698,-1.03927060553121,
-1.03235603928805,-1.02948599783301,-1.02769235386209,-1.02573127434595,
-1.02302660807084,-1.01661751513893,-0.988120778224044,-0.937199691808353,
-0.92570593998298,-0.923532784663462,-0.922168306560197,-0.921095644958398,
-0.919851398673143,-0.917634983655801,-0.907256255625866,-0.88479949620845,
-0.826425683167227,-0.820074640884895,-0.817579909948831,-0.815765546174149,
-0.813819997106104,-0.811204332633417,-0.805306067097214,-0.780904425918359,
-0.730243664865649,-0.714073288020118,-0.711447082232428,-0.710098342018559,
-0.70902691223935,-0.707771219535754,-0.705502142204713,-0.69425508762572,
-0.668580750836144,-0.615124095566524,-0.60826688100222,-0.605406389703567,
-0.603614565077583,-0.601652134216144,-0.598939470614618,-0.592482316776173,
-0.538648842451557,-0.502333043684892,-0.499481707201636,-0.498105350023912,
-0.497031682506023,-0.495795697428157,-0.493616772444554,-0.483806088750772,
-0.434911600178473,-0.39978588705918,-0.395498300221219,-0.392959320398786,
-0.391019040319279,-0.388944906261988,-0.38569233592946,-0.375347086631822,
-0.358709391730538,-0.325788065870077,-0.307647528961386,-0.2901527056505,
-0.287476521900033,-0.286117157539036,-0.285045058424708,-0.283797502071491,
-0.281565404343079,-0.270933199713164,-0.247567356259084,-0.191910477658296,
-0.184487386175552,-0.181531997981181,-0.179722854124052,-0.177893796424317,
-0.175383406597913,-0.170030959687916,-0.162914048401213,-0.145410500276712,
-0.0956238241308649,-0.0781599967756867,-0.0754850053838553,-0.0747630397369221),
 .UNSPECIFIED.);
#971=B_SPLINE_CURVE_WITH_KNOTS('',3,(#98175,#98176,#98177,#98178,#98179,
#98180,#98181,#98182,#98183,#98184,#98185,#98186,#98187,#98188,#98189,#98190,
#98191,#98192,#98193,#98194,#98195,#98196,#98197,#98198,#98199,#98200,#98201,
#98202,#98203,#98204,#98205,#98206,#98207,#98208,#98209,#98210,#98211,#98212,
#98213,#98214,#98215,#98216,#98217,#98218,#98219,#98220,#98221,#98222,#98223,
#98224,#98225,#98226,#98227,#98228,#98229,#98230,#98231,#98232,#98233,#98234,
#98235,#98236,#98237,#98238,#98239,#98240,#98241,#98242,#98243,#98244,#98245,
#98246,#98247,#98248,#98249,#98250,#98251,#98252,#98253,#98254,#98255,#98256,
#98257,#98258,#98259,#98260,#98261,#98262,#98263,#98264,#98265,#98266,#98267,
#98268,#98269,#98270,#98271,#98272,#98273,#98274,#98275,#98276,#98277,#98278,
#98279,#98280,#98281,#98282,#98283,#98284,#98285,#98286,#98287,#98288,#98289,
#98290,#98291,#98292,#98293,#98294,#98295,#98296,#98297,#98298,#98299,#98300,
#98301,#98302,#98303,#98304,#98305,#98306,#98307,#98308,#98309,#98310,#98311,
#98312,#98313,#98314,#98315,#98316,#98317,#98318,#98319,#98320,#98321,#98322,
#98323,#98324,#98325,#98326,#98327,#98328,#98329,#98330,#98331,#98332,#98333,
#98334,#98335,#98336,#98337,#98338,#98339,#98340,#98341,#98342,#98343,#98344,
#98345,#98346,#98347,#98348,#98349,#98350,#98351,#98352,#98353,#98354,#98355,
#98356,#98357,#98358,#98359,#98360,#98361,#98362,#98363,#98364,#98365,#98366,
#98367,#98368,#98369,#98370,#98371,#98372,#98373,#98374,#98375,#98376,#98377,
#98378,#98379,#98380,#98381,#98382,#98383,#98384,#98385,#98386,#98387,#98388,
#98389,#98390,#98391,#98392,#98393,#98394,#98395,#98396,#98397,#98398,#98399,
#98400,#98401,#98402,#98403,#98404,#98405,#98406,#98407,#98408,#98409,#98410,
#98411,#98412,#98413,#98414,#98415,#98416,#98417,#98418,#98419,#98420,#98421,
#98422,#98423,#98424,#98425,#98426,#98427,#98428,#98429,#98430,#98431,#98432,
#98433,#98434,#98435,#98436,#98437,#98438,#98439,#98440,#98441,#98442,#98443,
#98444),.UNSPECIFIED.,.F.,.F.,(4,2,2,2,2,2,2,2,2,2,2,2,2,2,2,2,2,2,2,2,
2,2,2,2,2,2,2,2,2,2,2,2,2,2,2,2,2,2,2,2,2,2,2,2,2,2,2,2,2,2,2,2,2,2,2,2,
2,2,2,2,2,2,2,2,2,2,2,2,2,2,2,2,2,2,2,2,2,2,2,2,2,2,2,2,2,2,2,2,2,2,2,2,
2,2,2,2,2,2,2,2,2,2,2,2,2,2,2,2,2,2,2,2,2,2,2,2,2,2,2,2,2,2,2,2,2,2,2,2,
2,2,2,2,2,2,4),(-2.59340742691029,-2.57482683816369,-2.55598428705709,-2.54668929628617,
-2.54454640880166,-2.54331827533432,-2.5422432615787,-2.54085440506306,
-2.53793953358015,-2.50824286242268,-2.45779351324169,-2.4483044705862,
-2.44369718445865,-2.43991807765489,-2.43774736955123,-2.43773167510825,
-2.43771542809484,-2.4376986083976,-2.43768119517003,-2.43766316681614,
-2.43764450094062,-2.43762517432277,-2.43760516292549,-2.43758444181548,
-2.43756298519575,-2.43754076634933,-2.43751775690632,-2.43749772062185,
-2.43747437033533,-2.43744716395983,-2.43741547348671,-2.43737857258338,
-2.43733562298907,-2.4372814105044,-2.43534068744899,-2.43279867369071,
-2.42850049441156,-2.39337894217525,-2.3444197610308,-2.33472076041937,
-2.33254960873209,-2.33131538333458,-2.33024155061225,-2.32886275572408,
-2.32599871442945,-2.29004668201088,-2.2572799032197,-2.23471839779757,
-2.22906471274651,-2.22649348217233,-2.22455509691613,-2.22272848071384,
-2.22018670929407,-2.21354621783687,-2.15773754627064,-2.13367776544556,
-2.12285518790877,-2.12061130091228,-2.11936109893463,-2.11828916558737,
-2.11693313448587,-2.11478757245249,-2.10375041867314,-2.05253448171894,
-2.02382498692971,-2.01739126118217,-2.01468258840941,-2.01272092541467,
-2.01092834882572,-2.00806348798411,-2.00117935327486,-1.94810328336587,
-1.9221968195101,-1.91088984480889,-1.9086173939238,-1.90736099249572,-1.90628966520143,
-1.90494194819707,-1.90232036973582,-1.8862782735189,-1.88098880635368,
-1.86640333575631,-1.83351148308965,-1.81694463870141,-1.80663224448225,
-1.80338329239783,-1.80130986038324,-1.79936911039311,-1.79682789202798,
-1.79253291967179,-1.75742112231489,-1.70851711837857,-1.69874599446692,
-1.69656973652486,-1.69533431009532,-1.69426052228391,-1.69288320993399,
-1.69002715620144,-1.66722999397125,-1.6116189146061,-1.59560714931515,
-1.59183766553623,-1.58964919152793,-1.58773499075694,-1.58536571962127,
-1.58173237867305,-1.56463564194741,-1.55656635629851,-1.52175568049127,
-1.49770632715769,-1.48688681590627,-1.48464320740332,-1.48339311050977,
-1.48232123638361,-1.4809652405832,-1.47830495576461,-1.46125129225894,
-1.44263945105813,-1.40968326605101,-1.39303804334902,-1.38269035032521,
-1.37943743122769,-1.37736318170756,-1.37542286917012,-1.37288395695056,
-1.36859676254284,-1.33401557331994,-1.27804985039277,-1.2737760250553,
-1.27210444939211,-1.27109242088845,-1.26999008544948,-1.26842516708966,
-1.2645126452046,-1.25985927748007),.UNSPECIFIED.);
#972=B_SPLINE_CURVE_WITH_KNOTS('',3,(#98450,#98451,#98452,#98453,#98454,
#98455,#98456,#98457,#98458,#98459,#98460,#98461,#98462,#98463,#98464,#98465,
#98466,#98467),.UNSPECIFIED.,.F.,.F.,(4,2,2,2,2,2,2,2,4),(-0.0751187452951849,
-0.0651105015072089,-0.0603738607788016,-0.0579480733093331,-0.056029062931303,
-0.0538783931757228,-0.0516516905968622,-0.0483298714381254,-0.000628983405359937),
 .UNSPECIFIED.);
#973=B_SPLINE_CURVE_WITH_KNOTS('',3,(#98468,#98469,#98470,#98471,#98472,
#98473,#98474,#98475,#98476,#98477,#98478,#98479,#98480,#98481,#98482,#98483,
#98484,#98485,#98486,#98487,#98488,#98489,#98490,#98491,#98492,#98493,#98494,
#98495,#98496,#98497,#98498,#98499,#98500,#98501,#98502,#98503,#98504,#98505,
#98506,#98507,#98508,#98509,#98510,#98511,#98512,#98513,#98514,#98515,#98516,
#98517,#98518,#98519,#98520,#98521,#98522,#98523,#98524,#98525,#98526,#98527,
#98528,#98529,#98530,#98531,#98532,#98533,#98534,#98535,#98536,#98537,#98538,
#98539,#98540,#98541,#98542,#98543,#98544,#98545,#98546,#98547,#98548,#98549,
#98550,#98551,#98552,#98553,#98554,#98555,#98556,#98557,#98558,#98559,#98560,
#98561,#98562,#98563,#98564,#98565,#98566,#98567,#98568,#98569,#98570,#98571,
#98572,#98573,#98574,#98575,#98576,#98577,#98578,#98579,#98580,#98581,#98582,
#98583,#98584,#98585,#98586,#98587,#98588,#98589,#98590,#98591,#98592,#98593,
#98594,#98595,#98596,#98597,#98598,#98599,#98600,#98601,#98602,#98603,#98604,
#98605,#98606,#98607,#98608,#98609,#98610,#98611,#98612,#98613,#98614,#98615,
#98616,#98617,#98618,#98619,#98620,#98621,#98622,#98623,#98624,#98625,#98626,
#98627,#98628,#98629,#98630,#98631,#98632,#98633,#98634,#98635,#98636,#98637,
#98638,#98639,#98640,#98641,#98642,#98643,#98644,#98645,#98646,#98647,#98648,
#98649,#98650,#98651,#98652,#98653,#98654,#98655,#98656,#98657,#98658,#98659,
#98660,#98661,#98662,#98663,#98664,#98665,#98666,#98667,#98668,#98669,#98670,
#98671,#98672,#98673,#98674,#98675,#98676,#98677,#98678,#98679,#98680,#98681,
#98682,#98683,#98684,#98685,#98686,#98687,#98688,#98689,#98690,#98691),
 .UNSPECIFIED.,.F.,.F.,(4,2,2,2,2,2,2,2,2,2,2,2,2,2,2,2,2,2,2,2,2,2,2,2,
2,2,2,2,2,2,2,2,2,2,2,2,2,2,2,2,2,2,2,2,2,2,2,2,2,2,2,2,2,2,2,2,2,2,2,2,
2,2,2,2,2,2,2,2,2,2,2,2,2,2,2,2,2,2,2,2,2,2,2,2,2,2,2,2,2,2,2,2,2,2,2,2,
2,2,2,2,2,2,2,2,2,2,2,2,2,2,2,4),(-2.66767968022051,-2.62472410100834,-2.62179024369457,
-2.62010753067188,-2.61860262187355,-2.61751100562116,-2.61648365454228,
-2.61473395702785,-2.60995915844497,-2.57250918240443,-2.55112176284539,
-2.52297042937878,-2.51633518659523,-2.51419561335918,-2.51210518020193,
-2.51017009822064,-2.50766688638814,-2.50350334361195,-2.47491290010697,
-2.44422701153071,-2.42038341354095,-2.40963328825848,-2.40740385203333,
-2.40614667163674,-2.4050751247499,-2.40372769735748,-2.40110834559491,
-2.38511092113857,-2.34084084869684,-2.3185744941839,-2.31018753941203,
-2.30409399604709,-2.30141111926008,-2.29945370777524,-2.29765499483361,
-2.29475830215823,-2.28768450447225,-2.23758434766355,-2.19964488815378,
-2.19607528994373,-2.19456697515733,-2.19347478825612,-2.19244841498421,
-2.19070363208749,-2.18596101022418,-2.146805627867,-2.09846332216771,-2.09206436586189,
-2.08936118732208,-2.08740017201908,-2.08560589113307,-2.08273330123238,
-2.07580466365126,-2.02329274066577,-1.99697702324215,-1.98556517737468,
-1.9832863475584,-1.98202838131569,-1.98095690832146,-1.97961051949116,
-1.97699596098488,-1.96109665887807,-1.96029238517123,-1.95152276698426,
-1.94394862944422,-1.91164747970902,-1.89280694214238,-1.88149571974595,
-1.87813645891381,-1.87603839440241,-1.87410579794032,-1.87161913833119,
-1.86751194760779,-1.84109148772073,-1.79881875014397,-1.78190721562362,
-1.77324496704892,-1.77114948301669,-1.76993173638218,-1.7688546328313,
-1.76747151336861,-1.76518747620935,-1.75161477006505,-1.7497906086826,
-1.70241721420444,-1.67144194092423,-1.66698993464138,-1.66465431397224,
-1.66274182562227,-1.66052685731025,-1.65673931567436,-1.64214487790029,
-1.62987934262549,-1.58946826330187,-1.57061452885678,-1.56131572211745,
-1.55917244129718,-1.55794416077477,-1.55686906942419,-1.55548018012948,
-1.55256547806248,-1.52372835638706,-1.48561706845735,-1.46809153475096,
-1.457350451559,-1.4540527827418,-1.45196837394869,-1.45003129225038,-1.44751476137409,
-1.44330550528578,-1.41283079708318,-1.40845787076926),.UNSPECIFIED.);
#974=B_SPLINE_CURVE_WITH_KNOTS('',3,(#98693,#98694,#98695,#98696,#98697,
#98698,#98699,#98700,#98701,#98702,#98703,#98704,#98705,#98706,#98707,#98708,
#98709,#98710,#98711,#98712,#98713,#98714,#98715,#98716,#98717,#98718,#98719,
#98720,#98721,#98722,#98723,#98724,#98725,#98726,#98727,#98728,#98729,#98730,
#98731,#98732,#98733,#98734,#98735,#98736,#98737,#98738,#98739,#98740,#98741,
#98742,#98743,#98744,#98745,#98746,#98747,#98748,#98749,#98750,#98751,#98752,
#98753,#98754,#98755,#98756,#98757,#98758,#98759,#98760,#98761,#98762,#98763,
#98764,#98765,#98766,#98767,#98768,#98769,#98770,#98771,#98772,#98773,#98774,
#98775,#98776,#98777,#98778,#98779,#98780,#98781,#98782,#98783,#98784,#98785,
#98786,#98787,#98788,#98789,#98790,#98791,#98792,#98793,#98794,#98795,#98796,
#98797,#98798,#98799,#98800,#98801,#98802,#98803,#98804,#98805,#98806,#98807,
#98808,#98809,#98810,#98811,#98812,#98813,#98814,#98815,#98816,#98817,#98818,
#98819,#98820,#98821,#98822,#98823,#98824,#98825,#98826,#98827,#98828,#98829,
#98830,#98831,#98832,#98833,#98834,#98835,#98836,#98837,#98838,#98839,#98840,
#98841,#98842,#98843,#98844,#98845,#98846,#98847,#98848,#98849,#98850,#98851,
#98852,#98853,#98854,#98855,#98856,#98857,#98858,#98859,#98860,#98861,#98862,
#98863,#98864,#98865,#98866,#98867,#98868,#98869,#98870,#98871,#98872,#98873,
#98874,#98875,#98876,#98877,#98878,#98879,#98880,#98881,#98882,#98883,#98884,
#98885,#98886,#98887,#98888,#98889,#98890,#98891,#98892,#98893,#98894,#98895,
#98896,#98897,#98898,#98899,#98900,#98901,#98902,#98903,#98904,#98905,#98906,
#98907,#98908,#98909,#98910,#98911,#98912,#98913,#98914,#98915,#98916,#98917,
#98918,#98919,#98920,#98921,#98922,#98923,#98924,#98925,#98926,#98927,#98928,
#98929,#98930,#98931,#98932,#98933,#98934,#98935,#98936,#98937,#98938,#98939,
#98940,#98941,#98942),.UNSPECIFIED.,.F.,.F.,(4,2,2,2,2,2,2,2,2,2,2,2,2,
2,2,2,2,2,2,2,2,2,2,2,2,2,2,2,2,2,2,2,2,2,2,2,2,2,2,2,2,2,2,2,2,2,2,2,2,
2,2,2,2,2,2,2,2,2,2,2,2,2,2,2,2,2,2,2,2,2,2,2,2,2,2,2,2,2,2,2,2,2,2,2,2,
2,2,2,2,2,2,2,2,2,2,2,2,2,2,2,2,2,2,2,2,2,2,2,2,2,2,2,2,2,2,2,2,2,2,2,2,
2,2,2,4),(-1.25985927748007,-1.2453003608062,-1.18892655397525,-1.17208144320606,
-1.16846473424463,-1.16610063855232,-1.16418684615964,-1.16199469799336,
-1.15820841068723,-1.14196185488026,-1.08448807431236,-1.07951541021613,
-1.06352987734088,-1.060911520986,-1.05956446632786,-1.05849314205298,-1.05723614299795,
-1.05496107222932,-1.04361003416923,-1.01752857920213,-0.964657620824425,
-0.957754797560903,-0.954886795420749,-0.953093601313664,-0.95113235145535,
-0.948426237280657,-0.942007982302704,-0.913433004698384,-0.862236989550861,
-0.851077062547889,-0.848923967992624,-0.847565636064483,-0.84649352601687,
-0.845245009891988,-0.843008844389658,-0.832313136909083,-0.808717538316708,
-0.752155396513283,-0.745589991140517,-0.743060124960592,-0.741236653797819,
-0.739296606699633,-0.736714622157358,-0.731002178634805,-0.708006887754293,
-0.67499115512056,-0.653966523574106,-0.639427645202852,-0.63709784681296,
-0.635701516337916,-0.63462303800303,-0.633413705604618,-0.6313549244533,
-0.623142962897156,-0.60752833142615,-0.565798520565196,-0.53711876354255,
-0.532953909722397,-0.530450790170106,-0.52851628812586,-0.526426985273519,
-0.523105135828782,-0.512136787100746,-0.494092608375872,-0.44394973431467,
-0.427599056526347,-0.424965865279674,-0.423615707203438,-0.422544286663548,
-0.421289917907758,-0.41902655374547,-0.407874729225503,-0.382567093742985,
-0.328586314515925,-0.321773694005278,-0.318920747300034,-0.317130423203263,
-0.31516702993929,-0.312448234169004,-0.305953518114173,-0.27673112699336,
-0.230070278103009,-0.215487915813216,-0.21295319667546,-0.211639178896181,
-0.210624518118271,-0.210616805287299,-0.210609243251825,-0.210601822977389,
-0.210594536107828,-0.210587374869379,-0.210580332097621,-0.210573401037422,
-0.210566575349115,-0.210559849132122,-0.210553216948067,-0.210546673528998,
-0.21054021396125,-0.210533833739875,-0.210527528431888,-0.210521294041483,
-0.210515126684568,-0.210509022608291,-0.210502978392329,-0.210496990703806,
-0.210491056335889,-0.210485172242678,-0.210479335624958,-0.2092168030889,
-0.206832087639687,-0.193334800688978,-0.157490929439518,-0.113371995598794,
-0.109091768114718,-0.106555067457512,-0.104615329130127,-0.10254060815884,
-0.0992846763182317,-0.0889080167813931,-0.0721999787376405,-0.0417595395179099,
-0.00539337765390236,-0.0019346342927621,-0.000864008595668716,-0.000629065984911949),
 .UNSPECIFIED.);
#975=B_SPLINE_CURVE_WITH_KNOTS('',3,(#98943,#98944,#98945,#98946,#98947,
#98948,#98949,#98950,#98951,#98952,#98953,#98954,#98955,#98956,#98957,#98958),
 .UNSPECIFIED.,.F.,.F.,(4,3,3,3,3,4),(-28.973780262141,-28.9662570488944,
-28.8628842312553,-28.7596459044043,-28.6565264336763,-28.6232427996483),
 .UNSPECIFIED.);
#976=B_SPLINE_CURVE_WITH_KNOTS('',3,(#98963,#98964,#98965,#98966,#98967,
#98968,#98969,#98970,#98971,#98972,#98973,#98974,#98975,#98976,#98977,#98978,
#98979,#98980,#98981,#98982,#98983,#98984,#98985,#98986,#98987,#98988,#98989,
#98990,#98991,#98992,#98993,#98994,#98995,#98996,#98997,#98998,#98999,#99000,
#99001,#99002,#99003,#99004,#99005,#99006,#99007,#99008,#99009,#99010,#99011,
#99012,#99013,#99014,#99015,#99016,#99017,#99018,#99019,#99020,#99021,#99022,
#99023,#99024,#99025,#99026,#99027,#99028,#99029,#99030,#99031,#99032,#99033,
#99034,#99035,#99036,#99037,#99038,#99039,#99040,#99041,#99042,#99043,#99044,
#99045,#99046,#99047,#99048,#99049,#99050,#99051,#99052,#99053,#99054,#99055,
#99056,#99057,#99058,#99059,#99060,#99061,#99062,#99063,#99064,#99065,#99066,
#99067,#99068,#99069,#99070,#99071,#99072,#99073,#99074,#99075,#99076,#99077,
#99078,#99079,#99080,#99081,#99082,#99083,#99084,#99085,#99086,#99087,#99088,
#99089,#99090,#99091,#99092,#99093,#99094,#99095,#99096,#99097,#99098,#99099,
#99100,#99101,#99102,#99103,#99104,#99105,#99106,#99107,#99108,#99109,#99110,
#99111,#99112,#99113,#99114,#99115,#99116,#99117,#99118,#99119,#99120,#99121,
#99122,#99123,#99124,#99125,#99126,#99127,#99128,#99129,#99130,#99131,#99132,
#99133,#99134,#99135,#99136,#99137,#99138,#99139,#99140,#99141,#99142,#99143,
#99144,#99145,#99146,#99147,#99148,#99149,#99150,#99151,#99152,#99153,#99154,
#99155,#99156,#99157,#99158,#99159,#99160,#99161,#99162,#99163,#99164,#99165,
#99166,#99167,#99168,#99169,#99170,#99171,#99172,#99173,#99174,#99175,#99176,
#99177,#99178,#99179,#99180,#99181,#99182,#99183,#99184,#99185,#99186,#99187,
#99188,#99189,#99190,#99191,#99192),.UNSPECIFIED.,.F.,.F.,(4,2,2,2,2,2,
2,2,2,2,2,2,2,2,2,2,2,2,2,2,2,2,2,2,2,2,2,2,2,2,2,2,2,2,2,2,2,2,2,2,2,2,
2,2,2,2,2,2,2,2,2,2,2,2,2,2,2,2,2,2,2,2,2,2,2,2,2,2,2,2,2,2,2,2,2,2,2,2,
2,2,2,2,2,2,2,2,2,2,2,2,2,2,2,2,2,2,2,2,2,2,2,2,2,2,2,2,2,2,2,2,2,2,2,2,
4),(-1.40850345617201,-1.36250451573646,-1.34494900943431,-1.33419481042488,
-1.33089575910889,-1.32881108876358,-1.32687418677182,-1.32431500164865,
-1.31872847952724,-1.31130510818259,-1.29270347500342,-1.24997538983778,
-1.2273474473027,-1.2244953107059,-1.22311867193607,-1.22204483400428,-1.22080870839955,
-1.2186296690159,-1.20882068857082,-1.15991605969471,-1.1247973117897,-1.1205016822107,
-1.11796017308648,-1.11601924660279,-1.11394566929914,-1.11069657869125,
-1.10038441161275,-1.0838208737984,-1.05095809007793,-1.03712981709347,
-1.03048063830151,-1.01500686837124,-1.01240980420473,-1.01106731386943,
-1.00999623450115,-1.0087355830341,-1.00644381478281,-0.99479749617328,
-0.967532404107712,-0.947347744839536,-0.912839856004122,-0.908553222099429,
-0.906014345009378,-0.904073877213896,-0.901999283978811,-0.898745452814007,
-0.888391612125599,-0.871735724992802,-0.838796771955161,-0.820073798500927,
-0.803159970223715,-0.800504776643279,-0.799149791750072,-0.798077894640733,
-0.796826831193154,-0.794579127428686,-0.783694889469947,-0.759403779996519,
-0.703900320938727,-0.697225379495664,-0.694678172334579,-0.692850075244814,
-0.69091234580841,-0.688345759397979,-0.682717600218909,-0.675223835433109,
-0.656363543322428,-0.62648896074036,-0.604932996834984,-0.590970469428296,
-0.588668080580198,-0.587279772315641,-0.586202302509577,-0.58498828096516,
-0.582908514771049,-0.574439457500337,-0.558088593267182,-0.515618639097743,
-0.488627341173812,-0.484506365326267,-0.482016079125526,-0.480083460080147,
-0.477988168978493,-0.474639431430082,-0.463420964140881,-0.444797703854754,
-0.416498823850429,-0.3794856425165,-0.376648347789939,-0.375274854288603,
-0.374201570617981,-0.37296393266865,-0.370777056715919,-0.361219425346794,
-0.312151972743189,-0.276986587383239,-0.272691408891711,-0.270150390471309,
-0.268209967617141,-0.266137053316455,-0.262889262446382,-0.252778637183708,
-0.236574052786764,-0.198328775589665,-0.16765233551806,-0.164739946623118,
-0.163351838190139,-0.162277199530957,-0.16104927574273,-0.159757267178105,
-0.155110071046882,-0.128864882825383,-0.106990878701804,-0.10555961659102,
-0.0751187452951849),.UNSPECIFIED.);
#977=B_SPLINE_CURVE_WITH_KNOTS('',3,(#99194,#99195,#99196,#99197,#99198,
#99199,#99200,#99201,#99202,#99203,#99204,#99205,#99206,#99207,#99208,#99209,
#99210,#99211,#99212,#99213,#99214,#99215,#99216,#99217,#99218,#99219,#99220,
#99221,#99222,#99223,#99224,#99225,#99226,#99227,#99228,#99229,#99230,#99231,
#99232,#99233,#99234,#99235,#99236,#99237,#99238,#99239,#99240,#99241,#99242,
#99243,#99244,#99245,#99246,#99247,#99248,#99249,#99250,#99251,#99252,#99253,
#99254,#99255,#99256,#99257,#99258,#99259,#99260,#99261,#99262,#99263,#99264,
#99265,#99266,#99267,#99268,#99269,#99270,#99271,#99272,#99273,#99274,#99275,
#99276,#99277,#99278,#99279,#99280,#99281,#99282,#99283,#99284,#99285,#99286,
#99287,#99288,#99289,#99290,#99291,#99292,#99293,#99294,#99295,#99296,#99297,
#99298,#99299,#99300,#99301,#99302,#99303,#99304,#99305,#99306,#99307,#99308,
#99309,#99310,#99311,#99312,#99313,#99314,#99315,#99316,#99317,#99318,#99319,
#99320,#99321,#99322,#99323,#99324,#99325,#99326,#99327,#99328,#99329,#99330,
#99331,#99332,#99333,#99334,#99335,#99336,#99337,#99338,#99339,#99340,#99341,
#99342,#99343,#99344,#99345,#99346,#99347,#99348,#99349,#99350,#99351,#99352,
#99353,#99354,#99355,#99356,#99357,#99358,#99359,#99360,#99361,#99362,#99363,
#99364,#99365,#99366,#99367,#99368,#99369,#99370,#99371,#99372,#99373,#99374),
 .UNSPECIFIED.,.F.,.F.,(4,3,3,3,3,3,3,3,3,3,3,3,3,3,3,3,3,3,3,3,3,3,3,3,
3,3,3,3,3,3,3,3,3,3,3,3,3,3,3,3,3,3,3,3,3,3,3,3,3,3,3,3,3,3,3,3,3,3,3,3,
4),(-28.6232427996483,-28.5202020671231,-28.4171817224122,-28.3141477780892,
-28.2110001872004,-28.1077864185769,-28.0043998212242,-27.9674205989325,
-27.8640258618991,-27.7607845797987,-27.6576646144213,-27.5546100462273,
-27.4515868378846,-27.3485609952273,-27.2454282284644,-27.1422391370698,
-27.0388671437033,-26.9685841489706,-26.8651894118465,-26.7619481296552,
-26.6588281641866,-26.5557735959015,-26.4527503874678,-26.3497245447197,
-26.2465917778669,-26.1434026863829,-26.0400306929286,-25.9697476990087,
-25.8663529620659,-25.7631116800558,-25.6599917147674,-25.5569371466617,
-25.4539139384065,-25.3508880958355,-25.2477553291568,-25.1445662378454,
-25.0411942445594,-24.9709112490469,-24.8675165120623,-24.764275230012,
-24.6611552646861,-24.5581006965446,-24.4550774882552,-24.3520516456517,
-24.2489188789435,-24.145729787604,-24.0423577942927,-23.972074799085,-23.8686800615147,
-23.7654387788756,-23.6623188129593,-23.5592642442267,-23.4562410353463,
-23.3532151921528,-23.2500824248602,-23.1468933329387,-23.0435213390553,
-22.9732383491231,-22.8444301460849,-22.71772832931,-22.6905949549614),
 .UNSPECIFIED.);
#978=B_SPLINE_CURVE_WITH_KNOTS('',3,(#99375,#99376,#99377,#99378),
 .UNSPECIFIED.,.F.,.F.,(4,4),(-22.6905949549614,-22.341147276672),
 .UNSPECIFIED.);
#979=B_SPLINE_CURVE_WITH_KNOTS('',3,(#99384,#99385,#99386,#99387,#99388,
#99389,#99390,#99391,#99392,#99393,#99394,#99395,#99396,#99397,#99398,#99399,
#99400,#99401,#99402,#99403),.UNSPECIFIED.,.F.,.F.,(4,2,2,2,2,2,2,2,2,4),
(-0.0747369786533256,-0.0746917043583635,-0.0441247850379056,-0.0412120543920209,
-0.0398238392008842,-0.0387491436130767,-0.0375211834199767,-0.0362291455859954,
-0.0342514142578872,-0.000628700708297845),.UNSPECIFIED.);
#980=B_SPLINE_CURVE_WITH_KNOTS('',3,(#99404,#99405,#99406,#99407,#99408,
#99409,#99410,#99411,#99412,#99413,#99414,#99415,#99416,#99417,#99418,#99419,
#99420,#99421,#99422,#99423,#99424,#99425,#99426,#99427,#99428,#99429,#99430,
#99431,#99432,#99433,#99434,#99435,#99436,#99437,#99438,#99439,#99440,#99441,
#99442,#99443,#99444,#99445,#99446,#99447,#99448,#99449,#99450,#99451,#99452,
#99453,#99454,#99455,#99456,#99457,#99458,#99459,#99460,#99461,#99462,#99463,
#99464,#99465,#99466,#99467,#99468,#99469,#99470,#99471,#99472,#99473,#99474,
#99475,#99476,#99477,#99478,#99479,#99480,#99481,#99482,#99483,#99484,#99485,
#99486,#99487,#99488,#99489,#99490,#99491,#99492,#99493,#99494,#99495,#99496,
#99497,#99498,#99499,#99500,#99501,#99502,#99503,#99504,#99505,#99506,#99507,
#99508,#99509,#99510,#99511,#99512,#99513,#99514,#99515,#99516,#99517,#99518,
#99519,#99520,#99521,#99522,#99523,#99524,#99525,#99526,#99527,#99528,#99529,
#99530,#99531,#99532,#99533,#99534,#99535,#99536,#99537,#99538,#99539,#99540,
#99541,#99542,#99543,#99544,#99545,#99546,#99547,#99548,#99549,#99550,#99551,
#99552,#99553,#99554,#99555,#99556,#99557,#99558,#99559,#99560,#99561,#99562,
#99563,#99564,#99565,#99566,#99567,#99568,#99569,#99570,#99571,#99572,#99573,
#99574,#99575,#99576,#99577,#99578,#99579,#99580,#99581,#99582,#99583,#99584,
#99585,#99586,#99587,#99588,#99589,#99590,#99591,#99592,#99593,#99594,#99595,
#99596,#99597,#99598,#99599,#99600,#99601,#99602,#99603,#99604,#99605,#99606,
#99607,#99608,#99609,#99610,#99611,#99612,#99613,#99614,#99615,#99616,#99617,
#99618,#99619,#99620,#99621,#99622,#99623),.UNSPECIFIED.,.F.,.F.,(4,2,2,
2,2,2,2,2,2,2,2,2,2,2,2,2,2,2,2,2,2,2,2,2,2,2,2,2,2,2,2,2,2,2,2,2,2,2,2,
2,2,2,2,2,2,2,2,2,2,2,2,2,2,2,2,2,2,2,2,2,2,2,2,2,2,2,2,2,2,2,2,2,2,2,2,
2,2,2,2,2,2,2,2,2,2,2,2,2,2,2,2,2,2,2,2,2,2,2,2,2,2,2,2,2,2,2,2,2,2,4),
(-2.66803233840665,-2.63756098231509,-2.61104504151717,-2.60487784634831,
-2.60221454463273,-2.60026071576239,-2.59845779291116,-2.5955376168873,
-2.58832279345047,-2.54292015830957,-2.52278906795612,-2.50657463302681,
-2.49817823291225,-2.49613083544029,-2.49490269536407,-2.49382769389884,
-2.4924388769836,-2.48952417197382,-2.4594875300262,-2.40817359987131,-2.39935615826286,
-2.39296017747777,-2.39025768383555,-2.38829695675368,-2.38650279568053,
-2.38363008350252,-2.37669952838482,-2.32423037013766,-2.29789168812594,
-2.28647459224803,-2.2841956462714,-2.28293774015966,-2.28186639356041,
-2.28052025914637,-2.27790647491917,-2.26202755774909,-2.25734580100041,
-2.21491157309143,-2.18434974916272,-2.17990944461745,-2.17757644393979,
-2.17566431249257,-2.17344774309271,-2.16965253765773,-2.15496801665183,
-2.1427186298469,-2.10720583685401,-2.08476940723062,-2.07439567095383,
-2.07217959453477,-2.07093541917591,-2.06986274847982,-2.06849815981428,
-2.06579801463128,-2.0476114225318,-2.02952941819104,-1.99679984642993,
-1.97430061116869,-1.96865496205343,-1.96608497612474,-1.96414654745937,
-1.96231916850218,-1.95977517649344,-1.95312195390438,-1.89741705405606,
-1.87328022634548,-1.86243622495129,-1.86019079897614,-1.85894014579244,
-1.85786807594353,-1.8565121932485,-1.85436746745846,-1.84334738178677,
-1.79204768598337,-1.76338076399131,-1.75695165432538,-1.75424351532098,
-1.75228172714543,-1.75048868410597,-1.74762231192975,-1.74073057730078,
-1.68773195233868,-1.66176214196635,-1.65043831385018,-1.64816464980308,
-1.64690786969298,-1.64583639677136,-1.64448872223772,-1.64186789011254,
-1.62584195655305,-1.62044596501797,-1.60594088498659,-1.57304501320094,
-1.55028833588863,-1.54460772337546,-1.54203121186659,-1.54009166988328,
-1.53826603501481,-1.53572894730415,-1.52912027839379,-1.472970285587,-1.44912112120558,
-1.43835460474416,-1.4361137768135,-1.43486407351235,-1.43379182328975,
-1.43243443547867,-1.42976867024961,-1.41258192057445,-1.40850345617201),
 .UNSPECIFIED.);
#981=B_SPLINE_CURVE_WITH_KNOTS('',3,(#99625,#99626,#99627,#99628,#99629,
#99630,#99631,#99632,#99633,#99634),.UNSPECIFIED.,.F.,.F.,(4,1,1,1,1,1,
1,4),(-22.341147276672,-21.9744018991612,-20.9755654491994,-19.9767289992375,
-18.9778925492756,-17.9790560993137,-16.9802196493519,-16.4074096477818),
 .UNSPECIFIED.);
#982=B_SPLINE_CURVE_WITH_KNOTS('',3,(#99635,#99636,#99637,#99638,#99639,
#99640),.UNSPECIFIED.,.F.,.F.,(4,2,4),(-2.66742168919182,-2.60891632325169,
-2.59315595175498),.UNSPECIFIED.);
#983=B_SPLINE_CURVE_WITH_KNOTS('',3,(#99645,#99646,#99647,#99648,#99649,
#99650,#99651,#99652,#99653,#99654,#99655,#99656,#99657,#99658,#99659,#99660,
#99661,#99662,#99663,#99664,#99665,#99666,#99667,#99668,#99669,#99670,#99671,
#99672,#99673,#99674,#99675,#99676,#99677,#99678,#99679,#99680,#99681,#99682,
#99683,#99684,#99685,#99686,#99687,#99688,#99689,#99690,#99691,#99692,#99693,
#99694,#99695,#99696,#99697,#99698,#99699,#99700,#99701,#99702,#99703,#99704,
#99705,#99706,#99707,#99708,#99709,#99710,#99711,#99712,#99713,#99714,#99715,
#99716,#99717,#99718,#99719,#99720,#99721,#99722,#99723,#99724,#99725,#99726,
#99727,#99728,#99729,#99730,#99731,#99732,#99733,#99734,#99735,#99736,#99737,
#99738,#99739,#99740,#99741,#99742,#99743,#99744,#99745,#99746,#99747,#99748,
#99749,#99750,#99751,#99752,#99753,#99754,#99755,#99756,#99757,#99758,#99759,
#99760,#99761,#99762,#99763,#99764,#99765,#99766,#99767,#99768,#99769,#99770,
#99771,#99772,#99773,#99774,#99775,#99776,#99777,#99778,#99779,#99780,#99781,
#99782,#99783,#99784,#99785,#99786,#99787,#99788,#99789,#99790,#99791,#99792,
#99793,#99794,#99795,#99796,#99797,#99798,#99799,#99800,#99801,#99802,#99803,
#99804,#99805,#99806,#99807,#99808,#99809,#99810,#99811,#99812,#99813,#99814,
#99815,#99816,#99817,#99818,#99819,#99820,#99821,#99822,#99823,#99824,#99825,
#99826,#99827,#99828,#99829,#99830,#99831,#99832,#99833,#99834,#99835,#99836,
#99837,#99838,#99839,#99840,#99841,#99842,#99843,#99844,#99845,#99846,#99847,
#99848,#99849,#99850,#99851,#99852,#99853,#99854,#99855,#99856,#99857,#99858,
#99859,#99860,#99861,#99862,#99863,#99864,#99865,#99866,#99867,#99868),
 .UNSPECIFIED.,.F.,.F.,(4,2,2,2,2,2,2,2,2,2,2,2,2,2,2,2,2,2,2,2,2,2,2,2,
2,2,2,2,2,2,2,2,2,2,2,2,2,2,2,2,2,2,2,2,2,2,2,2,2,2,2,2,2,2,2,2,2,2,2,2,
2,2,2,2,2,2,2,2,2,2,2,2,2,2,2,2,2,2,2,2,2,2,2,2,2,2,2,2,2,2,2,2,2,2,2,2,
2,2,2,2,2,2,2,2,2,2,2,2,2,2,2,4),(-1.40835994883514,-1.36496506558018,-1.33391364373284,
-1.31586282059911,-1.31316705999715,-1.31180334434074,-1.31073066522904,
-1.30948568806857,-1.30726626420923,-1.2968425515049,-1.27422806295316,
-1.21610121026393,-1.20971724338068,-1.20721686303649,-1.2054009159603,
-1.20345603859551,-1.20084540259578,-1.19497607013632,-1.17079842029402,
-1.12031274141491,-1.11988217351818,-1.10369440289438,-1.1010672943475,
-1.09971827769369,-1.0986467310789,-1.09739102239637,-1.0951222013546,-1.08388219691806,
-1.05823696210302,-1.0047299889714,-0.997875830436784,-0.995015684784422,
-0.993223806884562,-0.991261100244711,-0.988547655634353,-0.982086738624371,
-0.928142472106462,-0.891938229429457,-0.889083296460058,-0.887706160402034,
-0.886632335220905,-0.88539667680955,-0.883219546047789,-0.873437169264997,
-0.824513737505249,-0.789389722855819,-0.785094260725997,-0.782552881291843,
-0.780612071524827,-0.778538636076012,-0.775289803628643,-0.764978759501409,
-0.748417316710418,-0.715557434330294,-0.701818968594614,-0.694962270382339,
-0.694630896294975,-0.679575430470702,-0.677223593877109,-0.675820747720329,
-0.674741303903174,-0.673535405043201,-0.671492393166578,-0.66347021817228,
-0.648388371998441,-0.609029401102905,-0.577343038478701,-0.573108420984722,
-0.570584785065836,-0.568646917695049,-0.566566257155397,-0.563284255140809,
-0.552679768363485,-0.535463692706438,-0.488765062601624,-0.483699710436784,
-0.467678455037713,-0.465058089554265,-0.463710621449197,-0.462639295186871,
-0.461382672922729,-0.459109244683259,-0.447786119972239,-0.421813981997778,
-0.368788719256553,-0.361897881478697,-0.359031896395174,-0.357239102634568,
-0.355277598796495,-0.352569865805326,-0.346141767713424,-0.296439522833372,
-0.277531765598874,-0.271357445521186,-0.255652001523959,-0.253045247285455,
-0.251700742085052,-0.250629639458679,-0.249370802229852,-0.247132974643905,
-0.236261769431149,-0.211953870815406,-0.156483392049982,-0.149806229631321,
-0.147258804324013,-0.145430745588595,-0.143493235702129,-0.140927243534818,
-0.135301616819205,-0.116186404503192,-0.0947905862222214,-0.0747369786533256),
 .UNSPECIFIED.);
#984=B_SPLINE_CURVE_WITH_KNOTS('',3,(#99869,#99870,#99871,#99872,#99873,
#99874,#99875,#99876,#99877,#99878,#99879,#99880,#99881,#99882,#99883,#99884,
#99885,#99886,#99887,#99888,#99889,#99890,#99891,#99892,#99893,#99894,#99895,
#99896,#99897,#99898,#99899,#99900,#99901,#99902,#99903,#99904,#99905,#99906,
#99907,#99908,#99909,#99910,#99911,#99912,#99913,#99914,#99915,#99916,#99917,
#99918,#99919,#99920,#99921,#99922,#99923,#99924,#99925,#99926,#99927,#99928,
#99929,#99930,#99931,#99932,#99933,#99934,#99935,#99936,#99937,#99938,#99939,
#99940,#99941,#99942,#99943,#99944,#99945,#99946,#99947,#99948,#99949,#99950,
#99951,#99952,#99953,#99954,#99955,#99956,#99957,#99958,#99959,#99960,#99961,
#99962,#99963,#99964,#99965,#99966,#99967,#99968,#99969,#99970,#99971,#99972,
#99973,#99974,#99975,#99976,#99977,#99978,#99979,#99980,#99981,#99982,#99983,
#99984,#99985,#99986,#99987,#99988,#99989,#99990,#99991,#99992,#99993,#99994,
#99995,#99996,#99997,#99998,#99999,#100000,#100001,#100002,#100003,#100004,
#100005,#100006,#100007,#100008,#100009,#100010,#100011,#100012,#100013,
#100014,#100015,#100016,#100017,#100018,#100019,#100020,#100021,#100022,
#100023,#100024,#100025,#100026,#100027,#100028,#100029,#100030,#100031,
#100032,#100033,#100034,#100035,#100036,#100037,#100038,#100039,#100040,
#100041,#100042,#100043,#100044,#100045,#100046,#100047,#100048,#100049,
#100050,#100051,#100052,#100053,#100054,#100055,#100056,#100057,#100058,
#100059,#100060,#100061,#100062,#100063,#100064,#100065,#100066,#100067,
#100068,#100069,#100070,#100071,#100072,#100073,#100074,#100075,#100076,
#100077,#100078,#100079,#100080,#100081,#100082,#100083,#100084,#100085,
#100086,#100087,#100088,#100089,#100090,#100091,#100092,#100093,#100094,
#100095,#100096,#100097,#100098,#100099,#100100,#100101,#100102),
 .UNSPECIFIED.,.F.,.F.,(4,2,2,2,2,2,2,2,2,2,2,2,2,2,2,2,2,2,2,2,2,2,2,2,
2,2,2,2,2,2,2,2,2,2,2,2,2,2,2,2,2,2,2,2,2,2,2,2,2,2,2,2,2,2,2,2,2,2,2,2,
2,2,2,2,2,2,2,2,2,2,2,2,2,2,2,2,2,2,2,2,2,2,2,2,2,2,2,2,2,2,2,2,2,2,2,2,
2,2,2,2,2,2,2,2,2,2,2,2,2,2,2,2,2,2,2,2,4),(-2.59315595175498,-2.59007765275903,
-2.58078447923624,-2.57864198428897,-2.57741407158795,-2.57633924894897,
-2.57495063650189,-2.57203626622376,-2.54226190570917,-2.49162780586257,
-2.48229537460191,-2.47774308858225,-2.47500472226365,-2.47252035112126,
-2.47064426401568,-2.46881786361953,-2.46627671620563,-2.45963978199326,
-2.40381757790562,-2.37976765768529,-2.36894792452057,-2.3667042753065,
-2.36545415640015,-2.36438225645688,-2.36302622165248,-2.36088057815684,
-2.34984137340878,-2.29863196780722,-2.26992326006183,-2.26348974153481,
-2.26078115893801,-2.25881956202766,-2.25702704627416,-2.25416228338041,
-2.24727838555588,-2.19420739795661,-2.16829981453399,-2.15699274373935,
-2.15472035019834,-2.15346399068911,-2.15239271826015,-2.15104508986307,
-2.14842370921987,-2.13238317709358,-2.12707675461306,-2.11250768316067,
-2.07961731534741,-2.06305116899584,-2.05273924434692,-2.04949046792405,
-2.0474171553536,-2.04547652252956,-2.04293546559637,-2.03864078494573,
-2.00353525182107,-1.95465260835331,-1.94486020574292,-1.94268258638578,
-1.9414469068712,-1.94037323118513,-1.93899649901611,-1.93614315182974,
-1.9134506950524,-1.87272384866466,-1.8456806874179,-1.8394485375509,-1.83677416923669,
-1.83481856897838,-1.83301845087596,-1.8301126932048,-1.82298257636981,
-1.77422308648144,-1.735052660683,-1.7314780270815,-1.72996902053583,-1.72887685708661,
-1.72785086943613,-1.72610764747515,-1.72137451372362,-1.68180129920979,
-1.63388992385648,-1.62749311324278,-1.62479053644258,-1.62282984461181,
-1.62103578113662,-1.61816336611532,-1.61123424082424,-1.55875512132802,
-1.53242866751436,-1.52101503212502,-1.51873640125128,-1.51747861856325,
-1.51640744559843,-1.51506158295104,-1.51244823517107,-1.49656816267521,
-1.4906980547015,-1.44666701273634,-1.42810815161094,-1.41691845302898,
-1.41357286005854,-1.41147833449995,-1.40954560744237,-1.40705404760251,
-1.40292854603029,-1.37574265806748,-1.33373204506974,-1.32763511641381,
-1.30978754718718,-1.30709916290768,-1.30573723447465,-1.30466495342069,
-1.30341928442914,-1.3011958618825,-1.29070305756573,-1.26784057103001,
-1.2596092791427),.UNSPECIFIED.);
#985=B_SPLINE_CURVE_WITH_KNOTS('',3,(#100108,#100109,#100110,#100111,#100112,
#100113,#100114,#100115,#100116,#100117,#100118,#100119,#100120,#100121,
#100122,#100123,#100124,#100125,#100126,#100127,#100128,#100129,#100130,
#100131,#100132,#100133,#100134,#100135,#100136,#100137,#100138,#100139,
#100140,#100141,#100142,#100143,#100144,#100145,#100146,#100147,#100148,
#100149,#100150,#100151,#100152,#100153,#100154,#100155,#100156,#100157,
#100158,#100159,#100160,#100161,#100162,#100163,#100164,#100165,#100166,
#100167,#100168,#100169,#100170,#100171,#100172,#100173,#100174,#100175,
#100176,#100177,#100178,#100179,#100180,#100181,#100182,#100183,#100184,
#100185,#100186,#100187,#100188,#100189,#100190,#100191,#100192,#100193,
#100194,#100195,#100196,#100197,#100198,#100199,#100200,#100201,#100202,
#100203,#100204,#100205,#100206,#100207,#100208,#100209,#100210,#100211,
#100212,#100213),.UNSPECIFIED.,.F.,.F.,(4,3,3,3,3,3,3,3,3,3,3,3,3,3,3,3,
3,3,3,3,3,3,3,3,3,3,3,3,3,3,3,3,3,3,3,4),(-3.4905420523601,-3.38888724871603,
-3.2871461686745,-3.18536353037361,-3.08340260597814,-2.99650934988562,
-2.89298805351487,-2.78961775740443,-2.68636579627279,-2.58317747650148,
-2.48001897640827,-2.37685651582113,-2.27358608503739,-2.17025853571452,
-2.0667483835289,-1.99767289992375,-1.89536967835424,-1.79322051059792,
-1.69118874726443,-1.58921969074132,-1.48727797529671,-1.3853282756702,
-1.28325622478001,-1.18112117613606,-1.07878042700533,-0.998836449961875,
-0.892562662128034,-0.78099232936203,-0.675071864520977,-0.569250995903944,
-0.463501983636266,-0.357797177553288,-0.252079241114024,-0.146356223433945,
-0.0405602493167351,0.),.UNSPECIFIED.);
#986=B_SPLINE_CURVE_WITH_KNOTS('',3,(#100216,#100217,#100218,#100219,#100220,
#100221,#100222,#100223,#100224,#100225,#100226,#100227,#100228,#100229,
#100230,#100231,#100232,#100233,#100234,#100235,#100236,#100237,#100238,
#100239,#100240,#100241,#100242,#100243,#100244,#100245,#100246,#100247,
#100248,#100249,#100250,#100251,#100252,#100253,#100254,#100255,#100256,
#100257,#100258,#100259,#100260,#100261,#100262,#100263,#100264,#100265,
#100266,#100267,#100268,#100269,#100270,#100271,#100272,#100273,#100274,
#100275,#100276,#100277,#100278,#100279,#100280,#100281,#100282,#100283,
#100284,#100285,#100286,#100287,#100288,#100289,#100290,#100291,#100292,
#100293,#100294,#100295,#100296,#100297,#100298,#100299,#100300,#100301,
#100302,#100303,#100304,#100305,#100306,#100307,#100308,#100309,#100310,
#100311,#100312,#100313,#100314,#100315,#100316,#100317,#100318,#100319,
#100320,#100321,#100322,#100323,#100324,#100325,#100326,#100327,#100328,
#100329,#100330,#100331,#100332,#100333,#100334,#100335,#100336,#100337,
#100338,#100339,#100340,#100341,#100342,#100343,#100344,#100345,#100346,
#100347,#100348,#100349,#100350,#100351,#100352,#100353,#100354,#100355,
#100356,#100357,#100358,#100359,#100360,#100361,#100362,#100363,#100364,
#100365,#100366,#100367,#100368,#100369,#100370,#100371,#100372,#100373,
#100374,#100375),.UNSPECIFIED.,.F.,.F.,(4,3,3,3,3,3,3,3,3,3,3,3,3,3,3,3,
3,3,3,3,3,3,3,3,3,3,3,3,3,3,3,3,3,3,3,3,3,3,3,3,3,3,3,3,3,3,3,3,3,3,3,3,
3,4),(2.00878451797959,2.11210382153688,2.21526971314838,2.31831418782034,
2.42129345937127,2.5242416735564,2.62719293310596,2.73024899451787,2.83336205194682,
2.93665137518733,2.99650934988563,3.10008229381611,3.20350554280195,3.30681219802198,
3.4100562611044,3.51327148737704,3.61649159166828,3.71982072762219,3.82320766651887,
3.9267776968677,3.9953457998475,4.09860816546048,4.20171516905877,4.30469864795505,
4.40761543749366,4.51049977143292,4.61338583911078,4.71637840074732,4.81942682496838,
4.92265896654807,4.99418224980938,5.09760356589108,5.20087152694815,5.30401818826618,
5.40709944854827,5.51014930542219,5.61320171332603,5.71636073031365,5.81957593612848,
5.92297353214027,5.99301869977126,6.09643423322207,6.19969677808619,6.30283860095652,
6.40591538148351,6.50896112490232,6.61200979362757,6.71516567854846,6.81837808737287,
6.92177346211855,6.99185514973313,7.09672279961553,7.20139615639989,7.24304095782437),
 .UNSPECIFIED.);
#987=B_SPLINE_CURVE_WITH_KNOTS('',3,(#100381,#100382,#100383,#100384,#100385,
#100386,#100387,#100388,#100389,#100390,#100391,#100392,#100393,#100394,
#100395,#100396,#100397,#100398,#100399,#100400,#100401,#100402,#100403,
#100404,#100405,#100406),.UNSPECIFIED.,.F.,.F.,(4,2,2,2,2,2,2,2,2,2,2,2,
4),(-0.0747573277194267,-0.0739378941382004,-0.0616381618967872,-0.0559574691575537,
-0.0377855769967214,-0.0350634362630029,-0.0337175254258632,-0.032648440440134,
-0.0316335698164161,-0.0303960777140638,-0.0285521057197913,-0.0215326867205031,
-0.00065555548774641),.UNSPECIFIED.);
#988=B_SPLINE_CURVE_WITH_KNOTS('',3,(#100408,#100409,#100410,#100411,#100412,
#100413,#100414,#100415,#100416,#100417,#100418,#100419,#100420,#100421,
#100422,#100423,#100424,#100425,#100426,#100427,#100428,#100429,#100430,
#100431,#100432,#100433,#100434,#100435,#100436,#100437,#100438,#100439,
#100440,#100441,#100442,#100443,#100444,#100445,#100446,#100447,#100448,
#100449,#100450,#100451,#100452,#100453,#100454,#100455,#100456,#100457,
#100458,#100459,#100460,#100461,#100462,#100463,#100464,#100465,#100466,
#100467,#100468,#100469,#100470,#100471,#100472,#100473,#100474,#100475,
#100476,#100477,#100478,#100479,#100480,#100481,#100482,#100483,#100484,
#100485,#100486,#100487,#100488,#100489,#100490,#100491,#100492,#100493,
#100494,#100495,#100496,#100497,#100498,#100499,#100500,#100501,#100502,
#100503,#100504,#100505,#100506,#100507,#100508,#100509,#100510,#100511,
#100512,#100513,#100514,#100515,#100516,#100517,#100518,#100519,#100520,
#100521,#100522,#100523,#100524,#100525),.UNSPECIFIED.,.F.,.F.,(4,3,3,3,
3,3,3,3,3,3,3,3,3,3,3,3,3,3,3,3,3,3,3,3,3,3,3,3,3,3,3,3,3,3,3,3,3,3,3,4),
(170.955339710339,171.060905920727,171.162663399122,171.264353089028,171.366010721803,
171.467671980259,171.569433774519,171.671256094535,171.773239607341,171.799869393442,
171.903390392073,172.006760388742,172.110012049377,172.213200068173,172.316358267267,
172.419520427281,172.522790560255,172.626117812871,172.729627673424,172.798705843404,
172.901009665115,173.003159435031,173.105191801349,173.207161461353,173.309103780221,
173.411054082656,173.513126731748,173.615262377252,173.717603714352,173.797542293366,
173.903815640338,174.015386028212,174.121306049069,174.227126474861,174.332875046754,
174.43857941621,174.544296925171,174.650019520939,174.75581508523,174.796378743328),
 .UNSPECIFIED.);
#989=B_SPLINE_CURVE_WITH_KNOTS('',3,(#100529,#100530,#100531,#100532,#100533,
#100534,#100535,#100536,#100537,#100538,#100539,#100540,#100541,#100542,
#100543,#100544,#100545,#100546,#100547,#100548,#100549,#100550,#100551,
#100552,#100553,#100554,#100555,#100556,#100557,#100558,#100559,#100560,
#100561,#100562,#100563,#100564,#100565,#100566,#100567,#100568,#100569,
#100570,#100571,#100572,#100573,#100574,#100575,#100576,#100577,#100578,
#100579,#100580,#100581,#100582,#100583,#100584,#100585,#100586,#100587,
#100588,#100589,#100590,#100591,#100592,#100593,#100594,#100595,#100596,
#100597,#100598,#100599,#100600,#100601,#100602,#100603,#100604,#100605,
#100606,#100607,#100608,#100609,#100610,#100611,#100612,#100613,#100614,
#100615,#100616,#100617,#100618,#100619,#100620,#100621,#100622,#100623,
#100624,#100625,#100626,#100627,#100628,#100629,#100630,#100631,#100632,
#100633,#100634,#100635,#100636,#100637,#100638,#100639,#100640,#100641,
#100642,#100643,#100644,#100645,#100646,#100647,#100648,#100649,#100650,
#100651,#100652,#100653,#100654,#100655,#100656,#100657,#100658,#100659,
#100660,#100661,#100662,#100663,#100664,#100665,#100666,#100667,#100668,
#100669,#100670,#100671,#100672,#100673,#100674,#100675,#100676,#100677,
#100678,#100679,#100680,#100681,#100682,#100683,#100684,#100685,#100686,
#100687,#100688,#100689,#100690,#100691,#100692,#100693,#100694,#100695,
#100696,#100697),.UNSPECIFIED.,.F.,.F.,(4,3,3,3,3,3,3,3,3,3,3,3,3,3,3,3,
3,3,3,3,3,3,3,3,3,3,3,3,3,3,3,3,3,3,3,3,3,3,3,3,3,3,3,3,3,3,3,3,3,3,3,3,
3,3,3,3,4),(-172.787594225567,-172.684274861804,-172.581108909343,-172.478064373147,
-172.375085039686,-172.272136763294,-172.169185441327,-172.066129317591,
-171.963016197798,-171.859726812786,-171.799869393442,-171.696296438965,
-171.592873179124,-171.489566512639,-171.386322438044,-171.283107200028,
-171.179887083779,-171.076557935617,-170.973170984353,-170.869600941516,
-170.80103294348,-170.697770604844,-170.594663628611,-170.491680177536,
-170.388763416087,-170.285879110466,-170.182993071298,-170.080000538274,
-169.976952142771,-169.873720029761,-169.802196493519,-169.698775165844,
-169.595507193078,-169.492360519935,-169.389279247763,-169.286229378952,
-169.183176959081,-169.080017930163,-168.97680271242,-168.873405104616,
-168.803360043557,-168.69994450726,-168.59668195947,-168.493540133569,-168.390463349949,
-168.287417603378,-168.184368931446,-168.081213043256,-167.978000631122,
-167.874605253038,-167.804523593595,-167.699671753546,-167.594987925042,
-167.490464843253,-167.386036589514,-167.281667049056,-167.203857020092),
 .UNSPECIFIED.);
#990=B_SPLINE_CURVE_WITH_KNOTS('',3,(#100698,#100699,#100700,#100701,#100702,
#100703,#100704,#100705),.UNSPECIFIED.,.F.,.F.,(4,2,2,4),(-2.66736290127704,
-2.64532399614163,-2.59645533662874,-2.59317160363215),.UNSPECIFIED.);
#991=B_SPLINE_CURVE_WITH_KNOTS('',3,(#100710,#100711,#100712,#100713,#100714,
#100715,#100716,#100717,#100718,#100719,#100720,#100721,#100722,#100723,
#100724,#100725,#100726,#100727,#100728,#100729,#100730,#100731,#100732,
#100733,#100734,#100735,#100736,#100737,#100738,#100739,#100740,#100741,
#100742,#100743,#100744,#100745,#100746,#100747,#100748,#100749,#100750,
#100751,#100752,#100753,#100754,#100755,#100756,#100757,#100758,#100759,
#100760,#100761,#100762,#100763,#100764,#100765,#100766,#100767,#100768,
#100769,#100770,#100771,#100772,#100773,#100774,#100775,#100776,#100777,
#100778,#100779,#100780,#100781,#100782,#100783,#100784,#100785,#100786,
#100787,#100788,#100789,#100790,#100791,#100792,#100793,#100794,#100795,
#100796,#100797,#100798,#100799,#100800,#100801,#100802,#100803,#100804,
#100805,#100806,#100807,#100808,#100809,#100810,#100811,#100812,#100813,
#100814,#100815,#100816,#100817,#100818,#100819,#100820,#100821,#100822,
#100823,#100824,#100825,#100826,#100827,#100828,#100829,#100830,#100831,
#100832,#100833,#100834,#100835,#100836,#100837,#100838,#100839,#100840,
#100841,#100842,#100843,#100844,#100845,#100846,#100847,#100848,#100849,
#100850,#100851,#100852,#100853,#100854,#100855,#100856,#100857,#100858,
#100859,#100860,#100861,#100862,#100863,#100864,#100865,#100866,#100867,
#100868,#100869,#100870,#100871,#100872,#100873,#100874,#100875,#100876,
#100877,#100878,#100879,#100880,#100881,#100882,#100883,#100884,#100885,
#100886,#100887,#100888,#100889,#100890,#100891,#100892,#100893,#100894,
#100895,#100896,#100897,#100898,#100899,#100900,#100901,#100902,#100903,
#100904,#100905,#100906,#100907,#100908,#100909,#100910,#100911,#100912,
#100913,#100914,#100915,#100916,#100917,#100918,#100919,#100920,#100921,
#100922,#100923,#100924,#100925,#100926,#100927,#100928,#100929,#100930,
#100931,#100932,#100933,#100934,#100935),.UNSPECIFIED.,.F.,.F.,(4,2,2,2,
2,2,2,2,2,2,2,2,2,2,2,2,2,2,2,2,2,2,2,2,2,2,2,2,2,2,2,2,2,2,2,2,2,2,2,2,
2,2,2,2,2,2,2,2,2,2,2,2,2,2,2,2,2,2,2,2,2,2,2,2,2,2,2,2,2,2,2,2,2,2,2,2,
2,2,2,2,2,2,2,2,2,2,2,2,2,2,2,2,2,2,2,2,2,2,2,2,2,2,2,2,2,2,2,2,2,2,2,2,
4),(-1.4081797697387,-1.40705404714931,-1.40292854411527,-1.37574263943028,
-1.33373204743589,-1.32763514664634,-1.30978755123619,-1.3070991652891,
-1.30573723616672,-1.30466495463486,-1.30341928512133,-1.301195861737,-1.29070305468652,
-1.26784056022145,-1.21011173592253,-1.20367846621418,-1.20117010501504,
-1.19935224701617,-1.19740895594777,-1.19480674943785,-1.18898302718057,
-1.16514968570941,-1.11614973854379,-1.09779133429622,-1.09505199332823,
-1.09369780383667,-1.09262570304137,-1.09137328624521,-1.08912118833557,
-1.07817669697512,-1.05366058560861,-0.998557346910655,-0.991850158247918,
-0.989297544378724,-0.987467677688094,-0.985530001805971,-0.982966744492849,
-0.977359005991215,-0.929075125906758,-0.888723661534737,-0.884011299437307,
-0.882271324735715,-0.881246040259428,-0.880154604889832,-0.878645310963095,
-0.875062793117107,-0.870037675276166,-0.856213838582042,-0.833862609949703,
-0.787184867132219,-0.779989358286537,-0.777074355966871,-0.775273839853719,
-0.773322016017773,-0.770660377629352,-0.764492324022858,-0.737949806688716,
-0.698621228221383,-0.687287896511326,-0.673503643387962,-0.671211235544451,
-0.669826498440482,-0.668750047594006,-0.667534919431082,-0.665449594656343,
-0.656908206301732,-0.640348116914734,-0.598278238352605,-0.57109944187056,
-0.566971916353919,-0.564479092054117,-0.562545350303252,-0.560449685724274,
-0.55710216985586,-0.545904434824394,-0.527329229983804,-0.484804714632695,
-0.462028507280671,-0.459170643093303,-0.457791987418327,-0.456715722935139,
-0.455474742004388,-0.453287138242549,-0.443435079069284,-0.394232801530741,
-0.359839181976366,-0.355551477040888,-0.353009480827242,-0.351065107595321,
-0.348984818375656,-0.345718785888289,-0.335297078628961,-0.318505419793005,
-0.258883142282707,-0.249294128815231,-0.247244796286734,-0.245918179968781,
-0.244851141091832,-0.24384142056391,-0.241869026745214,-0.234451027456367,
-0.220917652702534,-0.192337636238333,-0.147271551995062,-0.143024731489448,
-0.14050666203384,-0.138580655494789,-0.136520215481735,-0.1332860526252,
-0.122977092776369,-0.106384522418824,-0.0845184776757566,-0.0747573277194267),
 .UNSPECIFIED.);
#992=B_SPLINE_CURVE_WITH_KNOTS('',3,(#100936,#100937,#100938,#100939,#100940,
#100941,#100942,#100943,#100944,#100945,#100946,#100947,#100948,#100949,
#100950,#100951,#100952,#100953,#100954,#100955,#100956,#100957,#100958,
#100959,#100960,#100961,#100962,#100963,#100964,#100965,#100966,#100967,
#100968,#100969,#100970,#100971,#100972,#100973,#100974,#100975,#100976,
#100977,#100978,#100979,#100980,#100981,#100982,#100983,#100984,#100985,
#100986,#100987,#100988,#100989,#100990,#100991,#100992,#100993,#100994,
#100995,#100996,#100997,#100998,#100999,#101000,#101001,#101002,#101003,
#101004,#101005,#101006,#101007,#101008,#101009,#101010,#101011,#101012,
#101013,#101014,#101015,#101016,#101017,#101018,#101019,#101020,#101021,
#101022,#101023,#101024,#101025,#101026,#101027,#101028,#101029,#101030,
#101031,#101032,#101033,#101034,#101035,#101036,#101037,#101038,#101039,
#101040,#101041,#101042,#101043,#101044,#101045,#101046,#101047,#101048,
#101049,#101050,#101051,#101052,#101053,#101054,#101055,#101056,#101057,
#101058,#101059,#101060,#101061,#101062,#101063,#101064,#101065,#101066,
#101067,#101068,#101069,#101070,#101071,#101072,#101073,#101074,#101075,
#101076,#101077,#101078,#101079,#101080,#101081,#101082,#101083,#101084,
#101085,#101086,#101087,#101088,#101089,#101090,#101091,#101092,#101093,
#101094,#101095,#101096,#101097,#101098,#101099,#101100,#101101,#101102,
#101103,#101104,#101105,#101106,#101107,#101108,#101109,#101110,#101111,
#101112,#101113,#101114,#101115,#101116,#101117,#101118,#101119,#101120,
#101121,#101122,#101123,#101124,#101125,#101126,#101127,#101128,#101129,
#101130,#101131,#101132,#101133,#101134,#101135,#101136,#101137,#101138,
#101139,#101140,#101141,#101142,#101143,#101144,#101145,#101146,#101147,
#101148,#101149,#101150,#101151,#101152,#101153,#101154,#101155,#101156,
#101157,#101158,#101159,#101160,#101161,#101162,#101163,#101164,#101165,
#101166,#101167,#101168,#101169,#101170,#101171,#101172,#101173,#101174,
#101175),.UNSPECIFIED.,.F.,.F.,(4,2,2,2,2,2,2,2,2,2,2,2,2,2,2,2,2,2,2,2,
2,2,2,2,2,2,2,2,2,2,2,2,2,2,2,2,2,2,2,2,2,2,2,2,2,2,2,2,2,2,2,2,2,2,2,2,
2,2,2,2,2,2,2,2,2,2,2,2,2,2,2,2,2,2,2,2,2,2,2,2,2,2,2,2,2,2,2,2,2,2,2,2,
2,2,2,2,2,2,2,2,2,2,2,2,2,2,2,2,2,2,2,2,2,2,2,2,2,2,2,4),(-2.59317160363215,
-2.58673594885869,-2.5845650297111,-2.5833317076338,-2.58225834819646,-2.58088032048256,
-2.57802034512731,-2.5419520152714,-2.50922401730088,-2.49284808246887,
-2.48605327914976,-2.48242696514828,-2.47932638804408,-2.47731985469502,
-2.47537866641607,-2.47283720339729,-2.46854251759948,-2.43358181895235,
-2.38476481586845,-2.37483908478156,-2.37265165323965,-2.37141340106578,
-2.37033969954126,-2.36896559378469,-2.3667606918179,-2.3547091910955,-2.35183965736574,
-2.34965884917676,-2.30370989443497,-2.2758044003634,-2.26946736754952,
-2.26677514184139,-2.26481648830571,-2.26302050320473,-2.26013671425176,
-2.25313750149361,-2.20171508737932,-2.1746326890419,-2.16303119512499,
-2.16074228671133,-2.15948241638636,-2.15841156517565,-2.15706880089489,
-2.15446949392708,-2.13893283302613,-2.13230550553906,-2.1184955936798,
-2.08561373455522,-2.06905687058442,-2.05874943017676,-2.05550143297457,
-2.05342846997416,-2.05148806203009,-2.04894715383983,-2.04465240459036,
-2.00951436769706,-1.9605727969908,-1.95086005968978,-1.94868809347177,
-1.94745375857685,-1.94637995106671,-1.94500141691688,-1.94213896761604,
-1.91877979985089,-1.90648241058348,-1.87361338966278,-1.85707369761816,
-1.84677342475686,-1.84352574329631,-1.84145250701174,-1.8395115070941,
-1.83696933507209,-1.83267134101501,-1.797329041018,-1.74815524971566,-1.73883781275927,
-1.73669328523529,-1.73546477758897,-1.73438985462556,-1.73300162788225,
-1.73008976366529,-1.69805880582034,-1.66514626925938,-1.64631885454103,
-1.63883435206517,-1.63321196328138,-1.63064632194556,-1.62870861843629,
-1.6268800432745,-1.62433136160931,-1.61764757677461,-1.56225455513589,
-1.53791207396448,-1.52701304662379,-1.52476438780703,-1.52351307202462,
-1.52244113574071,-1.52108632253533,-1.51843212865549,-1.50154965032546,
-1.48276192697767,-1.44979585562423,-1.43314256746031,-1.4227907804727,
-1.41953707096079,-1.41746243701401,-1.41552184894916,-1.41298269759226,
-1.40869537185761,-1.3649344835269,-1.33388337229201,-1.3158327292564,-1.31313699566266,
-1.31177329368198,-1.31070062533052,-1.30945566066131,-1.30723625909767,
-1.29681265159966,-1.27419839242439,-1.2597140489769),.UNSPECIFIED.);
#993=B_SPLINE_CURVE_WITH_KNOTS('',3,(#101181,#101182,#101183,#101184),
 .UNSPECIFIED.,.F.,.F.,(4,4),(158.039785877565,158.388969095546),
 .UNSPECIFIED.);
#994=B_SPLINE_CURVE_WITH_KNOTS('',3,(#101185,#101186,#101187,#101188,#101189,
#101190,#101191,#101192,#101193,#101194,#101195,#101196,#101197,#101198,
#101199,#101200,#101201,#101202,#101203,#101204,#101205,#101206,#101207,
#101208,#101209,#101210,#101211,#101212,#101213,#101214,#101215,#101216,
#101217,#101218,#101219,#101220,#101221,#101222,#101223,#101224,#101225,
#101226,#101227,#101228,#101229,#101230,#101231,#101232,#101233,#101234,
#101235,#101236,#101237,#101238,#101239,#101240,#101241,#101242,#101243,
#101244,#101245,#101246,#101247,#101248,#101249,#101250,#101251,#101252,
#101253,#101254,#101255,#101256,#101257,#101258,#101259,#101260,#101261,
#101262,#101263,#101264,#101265,#101266,#101267,#101268,#101269,#101270,
#101271,#101272,#101273,#101274,#101275,#101276,#101277,#101278,#101279,
#101280,#101281,#101282,#101283,#101284,#101285,#101286,#101287,#101288,
#101289,#101290,#101291,#101292,#101293,#101294,#101295,#101296,#101297,
#101298,#101299,#101300,#101301,#101302,#101303,#101304,#101305,#101306,
#101307,#101308,#101309,#101310,#101311,#101312,#101313,#101314,#101315,
#101316,#101317,#101318,#101319,#101320,#101321,#101322,#101323,#101324,
#101325,#101326,#101327,#101328,#101329,#101330,#101331,#101332,#101333,
#101334,#101335,#101336,#101337,#101338,#101339,#101340,#101341,#101342,
#101343,#101344,#101345,#101346,#101347,#101348,#101349,#101350,#101351,
#101352,#101353,#101354,#101355,#101356,#101357,#101358,#101359,#101360,
#101361,#101362,#101363,#101364,#101365,#101366,#101367,#101368,#101369,
#101370,#101371,#101372,#101373,#101374,#101375,#101376,#101377,#101378,
#101379,#101380,#101381,#101382,#101383,#101384,#101385,#101386,#101387,
#101388,#101389,#101390,#101391,#101392,#101393,#101394),.UNSPECIFIED.,
 .F.,.F.,(4,2,2,2,2,2,2,2,2,2,2,2,2,2,2,2,2,2,2,2,2,2,2,2,2,2,2,2,2,2,2,
2,2,2,2,2,2,2,2,2,2,2,2,2,2,2,2,2,2,2,2,2,2,2,2,2,2,2,2,2,2,2,2,2,2,2,2,
2,2,2,2,2,2,2,2,2,2,2,2,2,2,2,2,2,2,2,2,2,2,2,2,2,2,2,2,2,2,2,2,2,2,2,2,
2,4),(-2.66742167008063,-2.60891629962728,-2.59007761065181,-2.58078442973836,
-2.57864193350201,-2.57741402012589,-2.57633919693135,-2.57495058380529,
-2.57203621224051,-2.54225956113033,-2.49161991202839,-2.48229185293,-2.47774109911341,
-2.47500336193923,-2.47251944209562,-2.47064342803993,-2.46881688570725,
-2.46627520269848,-2.45963485678475,-2.40384585222558,-2.37977416007561,
-2.36894855197089,-2.36670454612067,-2.36545434923538,-2.36438245688096,
-2.36302652716526,-2.36088122886156,-2.34984760239113,-2.29862707678893,
-2.26992251375875,-2.26348948834143,-2.2607809886947,-2.25881940662941,
-2.25702687333504,-2.25416201476092,-2.24727753653619,-2.19421412030655,
-2.16830126967926,-2.15699285514878,-2.15472038412511,-2.15346400766958,
-2.15239273648127,-2.15104512962614,-2.14842384973225,-2.13238492277097,
-2.12706803551359,-2.11250738276455,-2.07961711069569,-2.06305108067805,
-2.05273920819065,-2.04949043734406,-2.04741712571751,-2.04547649193833,
-2.04293543109895,-2.03864073788547,-2.00353429981958,-1.9546488601183,
-1.94485976310371,-1.94268236885225,-1.9414467386515,-1.94037305564743,
-1.93899624853643,-1.93614252076347,-1.91343456440615,-1.87271784828833,
-1.8456797686759,-1.83944824396967,-1.8367739831557,-1.83481840150778,-1.83301825861359,
-1.83011236786878,-1.8229814589106,-1.77424216796041,-1.73505278561684,
-1.73147806347431,-1.72996904168253,-1.72887687551966,-1.72785089206481,
-1.72610769136682,-1.72137469754077,-1.68178582082112,-1.63388987681075,
-1.62749309848966,-1.62479052709872,-1.62282983619091,-1.62103577149068,
-1.61816334999122,-1.61123418574533,-1.55875561383704,-1.53242877602031,
-1.52101504363046,-1.51873640706946,-1.5174786230623,-1.51640744990724,
-1.51506158825751,-1.51244824645225,-1.49656843867832,-1.49069774516136,
-1.44666703398199,-1.42810816110467,-1.41691845656588,-1.41357286214017,
-1.41147833572777,-1.40954560791717,-1.4081797697387),.UNSPECIFIED.);
#995=B_SPLINE_CURVE_WITH_KNOTS('',3,(#101396,#101397,#101398,#101399,#101400,
#101401,#101402,#101403,#101404,#101405,#101406,#101407,#101408,#101409,
#101410,#101411,#101412,#101413,#101414,#101415,#101416,#101417,#101418,
#101419,#101420,#101421,#101422,#101423,#101424,#101425,#101426,#101427,
#101428,#101429,#101430,#101431,#101432,#101433,#101434,#101435,#101436,
#101437,#101438,#101439,#101440,#101441,#101442,#101443,#101444,#101445,
#101446,#101447,#101448,#101449,#101450,#101451,#101452,#101453,#101454,
#101455,#101456,#101457,#101458,#101459,#101460,#101461,#101462,#101463,
#101464,#101465,#101466,#101467,#101468,#101469,#101470,#101471,#101472,
#101473,#101474,#101475,#101476,#101477,#101478,#101479,#101480,#101481,
#101482,#101483,#101484,#101485,#101486,#101487,#101488,#101489,#101490,
#101491,#101492,#101493,#101494,#101495,#101496,#101497,#101498,#101499,
#101500,#101501,#101502,#101503,#101504,#101505,#101506,#101507,#101508,
#101509,#101510,#101511,#101512,#101513,#101514,#101515,#101516,#101517,
#101518,#101519,#101520,#101521,#101522,#101523,#101524,#101525,#101526,
#101527,#101528,#101529,#101530,#101531,#101532,#101533,#101534,#101535,
#101536,#101537,#101538,#101539,#101540,#101541,#101542,#101543,#101544,
#101545,#101546,#101547,#101548,#101549,#101550,#101551,#101552,#101553,
#101554,#101555,#101556,#101557,#101558,#101559,#101560,#101561,#101562,
#101563,#101564,#101565,#101566,#101567,#101568,#101569,#101570,#101571,
#101572,#101573,#101574,#101575,#101576,#101577,#101578,#101579,#101580,
#101581,#101582,#101583,#101584,#101585,#101586,#101587,#101588,#101589,
#101590,#101591,#101592,#101593,#101594,#101595,#101596,#101597,#101598,
#101599,#101600,#101601,#101602,#101603,#101604,#101605,#101606,#101607,
#101608,#101609,#101610,#101611,#101612,#101613,#101614,#101615),
 .UNSPECIFIED.,.F.,.F.,(4,2,2,2,2,2,2,2,2,2,2,2,2,2,2,2,2,2,2,2,2,2,2,2,
2,2,2,2,2,2,2,2,2,2,2,2,2,2,2,2,2,2,2,2,2,2,2,2,2,2,2,2,2,2,2,2,2,2,2,2,
2,2,2,2,2,2,2,2,2,2,2,2,2,2,2,2,2,2,2,2,2,2,2,2,2,2,2,2,2,2,2,2,2,2,2,2,
2,2,2,2,2,2,2,2,2,2,2,2,2,4),(-1.2597140489769,-1.21607211528067,-1.20968821294619,
-1.20718785775925,-1.20537192891124,-1.20342707102829,-1.20081646110999,
-1.19494718699638,-1.17076977582703,-1.12028459477336,-1.11985386727793,
-1.10366642251781,-1.10103934686962,-1.0996903451474,-1.09861880936702,
-1.09736311219612,-1.09509430894122,-1.08385433159205,-1.05820902126195,
-1.00470306390945,-0.997848935069586,-0.994988811669736,-0.993196950575264,
-0.991234264652791,-0.988520852931581,-0.982060034472249,-0.92811745660486,
-0.891912320049524,-0.889057454449225,-0.887680339810928,-0.886606526123829,
-0.885370875058493,-0.883193743168925,-0.873411128174183,-0.824488470402741,
-0.789364897809759,-0.78506947991398,-0.782528126301392,-0.780587336052889,
-0.778513921261863,-0.775265120777778,-0.764954174695253,-0.748392886195722,
-0.715533323037496,-0.701794094173061,-0.694939612471293,-0.69461438418154,
-0.688842051763052,-0.67901965223504,-0.676953893648946,-0.67562233210618,
-0.674551906554244,-0.673282549028711,-0.670950228963651,-0.658540221382086,
-0.602513479399798,-0.590215587091273,-0.575773210169352,-0.572000034767057,
-0.569788814639537,-0.567876739441582,-0.565538064780693,-0.561069247707397,
-0.529402403398003,-0.47805594926497,-0.467142212211925,-0.465004477830096,
-0.463650883099023,-0.462579200846446,-0.46132736876167,-0.459075726460668,
-0.4481227157292,-0.423571979107512,-0.368469533977642,-0.361757421964373,
-0.359204665749231,-0.357375232913841,-0.35543851228173,-0.352877366578463,
-0.347277710026164,-0.299799126900656,-0.280776151537551,-0.269754809606278,
-0.255489406696663,-0.253171642777262,-0.25177886671696,-0.250700886812702,
-0.249489600435585,-0.247463445738442,-0.239553872277646,-0.224727841231445,
-0.194394572833513,-0.183546222816926,-0.153290477246828,-0.149087099863418,
-0.146572705682888,-0.144636451558391,-0.142552127382758,-0.139252874556893,
-0.128491248907085,-0.0984667337296311,-0.0750459545985775,-0.0441238008826357,
-0.0412117068555677,-0.0398236153055869,-0.0387489326831677,-0.0375208947387947,
-0.0362287461449151,-0.0342507474909926,-0.000628701088768321),
 .UNSPECIFIED.);
#996=B_SPLINE_CURVE_WITH_KNOTS('',3,(#101616,#101617,#101618,#101619,#101620,
#101621,#101622,#101623,#101624,#101625,#101626,#101627,#101628,#101629,
#101630,#101631,#101632,#101633),.UNSPECIFIED.,.F.,.F.,(4,2,2,2,2,2,2,2,
4),(-2.66802706317801,-2.63755579499735,-2.6110399285369,-2.60487275085818,
-2.60220945676248,-2.60025563350888,-2.59845271585941,-2.59553254830194,
-2.59354406257328),.UNSPECIFIED.);
#997=B_SPLINE_CURVE_WITH_KNOTS('',3,(#101639,#101640,#101641,#101642,#101643,
#101644,#101645,#101646,#101647,#101648,#101649,#101650,#101651),
 .UNSPECIFIED.,.F.,.F.,(4,3,3,3,4),(151.755345484905,151.823140394205,151.951948597258,
152.078650414044,152.105783788367),.UNSPECIFIED.);
#998=B_SPLINE_CURVE_WITH_KNOTS('',3,(#101652,#101653,#101654,#101655,#101656,
#101657,#101658,#101659,#101660,#101661),.UNSPECIFIED.,.F.,.F.,(4,1,1,1,
1,1,1,4),(152.105783788367,152.821976844167,153.820813294129,154.81964974409,
155.818486194052,156.817322644014,157.816159093976,158.039785877565),
 .UNSPECIFIED.);
#999=B_SPLINE_CURVE_WITH_KNOTS('',3,(#101662,#101663,#101664,#101665,#101666,
#101667,#101668,#101669,#101670,#101671,#101672,#101673,#101674,#101675,
#101676,#101677,#101678,#101679,#101680,#101681,#101682,#101683,#101684,
#101685,#101686,#101687,#101688,#101689,#101690,#101691,#101692,#101693,
#101694,#101695,#101696,#101697,#101698,#101699,#101700,#101701,#101702,
#101703,#101704,#101705,#101706,#101707,#101708,#101709,#101710,#101711,
#101712,#101713,#101714,#101715,#101716,#101717,#101718,#101719,#101720,
#101721,#101722,#101723,#101724,#101725,#101726,#101727,#101728,#101729,
#101730,#101731,#101732,#101733,#101734,#101735,#101736,#101737,#101738,
#101739,#101740,#101741,#101742,#101743,#101744,#101745,#101746,#101747,
#101748,#101749,#101750,#101751,#101752,#101753,#101754,#101755,#101756,
#101757,#101758,#101759,#101760,#101761,#101762,#101763,#101764,#101765,
#101766,#101767,#101768,#101769,#101770,#101771,#101772,#101773,#101774,
#101775,#101776,#101777,#101778,#101779,#101780,#101781,#101782,#101783,
#101784,#101785,#101786,#101787,#101788,#101789,#101790,#101791,#101792,
#101793,#101794,#101795,#101796,#101797,#101798,#101799,#101800,#101801,
#101802,#101803,#101804,#101805,#101806,#101807,#101808,#101809,#101810,
#101811,#101812,#101813,#101814,#101815,#101816,#101817,#101818,#101819,
#101820,#101821,#101822,#101823,#101824,#101825,#101826,#101827,#101828,
#101829,#101830,#101831,#101832,#101833,#101834,#101835,#101836,#101837,
#101838,#101839,#101840,#101841,#101842,#101843,#101844,#101845,#101846,
#101847,#101848,#101849,#101850,#101851,#101852,#101853,#101854,#101855,
#101856,#101857,#101858,#101859,#101860,#101861,#101862,#101863,#101864,
#101865,#101866,#101867,#101868,#101869,#101870,#101871,#101872,#101873,
#101874,#101875,#101876,#101877,#101878,#101879,#101880,#101881,#101882,
#101883,#101884,#101885,#101886,#101887),.UNSPECIFIED.,.F.,.F.,(4,2,2,2,
2,2,2,2,2,2,2,2,2,2,2,2,2,2,2,2,2,2,2,2,2,2,2,2,2,2,2,2,2,2,2,2,2,2,2,2,
2,2,2,2,2,2,2,2,2,2,2,2,2,2,2,2,2,2,2,2,2,2,2,2,2,2,2,2,2,2,2,2,2,2,2,2,
2,2,2,2,2,2,2,2,2,2,2,2,2,2,2,2,2,2,2,2,2,2,2,2,2,2,2,2,2,2,2,2,2,2,2,2,
4),(-2.59354406257328,-2.5883177459959,-2.54291518852348,-2.52278407067703,
-2.50656977869565,-2.49817343625599,-2.49612604437296,-2.49489790920737,
-2.49382291060779,-2.49243409550616,-2.48951938763106,-2.45949266919019,
-2.40820649761714,-2.39936841407381,-2.39296073321018,-2.39025626196916,
-2.38829518038734,-2.386501439532,-2.38363102425653,-2.37671440318338,-2.32405266885479,
-2.29784933746303,-2.2864663988119,-2.2841894000465,-2.28293191795009,-2.28186053829543,
-2.28051386102173,-2.27789755233361,-2.26195311050385,-2.25752854000568,
-2.21497262544489,-2.18434770593607,-2.17990567312237,-2.17757231460419,
-2.17566016954263,-2.1734438994608,-2.16964997745239,-2.15497992752818,
-2.14272828679887,-2.10721337497845,-2.08476765647976,-2.07439129612995,
-2.07217505637237,-2.07093084721443,-2.06985818362316,-2.06849365084788,
-2.06579375923465,-2.04761477729643,-2.02952730104136,-1.99679696032674,
-1.97429645626121,-1.96865064186295,-1.96608062944405,-1.96414220066034,
-1.96231483619869,-1.95977088783293,-1.95311792005538,-1.89741077955412,
-1.87327558196273,-1.86243203046014,-1.8601866357617,-1.85893599134058,
-1.85786392366942,-1.85650803689063,-1.85436329183246,-1.84334283559094,
-1.79204287119749,-1.76337674192956,-1.75694773443749,-1.75423961683647,
-1.75227783631072,-1.75048479485884,-1.74761841346347,-1.74072659576553,
-1.68772942145559,-1.66175876004346,-1.65043472724724,-1.64816105561119,
-1.64690427580808,-1.64583280588096,-1.64448513859455,-1.64186433079932,
-1.62583873355727,-1.62044137963091,-1.60593735479828,-1.57304157782815,
-1.55028497605359,-1.54460438040687,-1.54202787592298,-1.540088338975,-1.53826270866202,
-1.53572562698701,-1.52911697206969,-1.47296714800935,-1.44911802646067,
-1.43835153256407,-1.43611071006738,-1.43486100990112,-1.43378876243328,
-1.43243137819505,-1.42976562024144,-1.4125789269329,-1.36250163812305,
-1.34494617418748,-1.33419200155471,-1.33089295855992,-1.32880829352727,
-1.32687139650913,-1.32431221801367,-1.3187257105899,-1.31130235891606,
-1.29270077583319,-1.25985604642124),.UNSPECIFIED.);
#1000=B_SPLINE_CURVE_WITH_KNOTS('',3,(#101893,#101894,#101895,#101896,#101897,
#101898,#101899,#101900,#101901,#101902,#101903,#101904,#101905,#101906),
 .UNSPECIFIED.,.F.,.F.,(4,2,2,2,2,2,4),(-0.0749180422499143,-0.0725023883060536,
-0.0418724803977279,-0.00539538322887077,-0.00193513678409589,-0.000864203141083117,
-0.000629064338207634),.UNSPECIFIED.);
#1001=B_SPLINE_CURVE_WITH_KNOTS('',3,(#101907,#101908,#101909,#101910,#101911,
#101912,#101913,#101914,#101915,#101916,#101917,#101918,#101919,#101920,
#101921,#101922,#101923,#101924,#101925,#101926,#101927,#101928,#101929,
#101930,#101931,#101932,#101933,#101934,#101935,#101936,#101937,#101938,
#101939,#101940,#101941,#101942,#101943,#101944,#101945,#101946,#101947,
#101948,#101949,#101950,#101951,#101952,#101953,#101954,#101955,#101956,
#101957,#101958,#101959,#101960,#101961,#101962,#101963,#101964,#101965,
#101966,#101967,#101968,#101969,#101970,#101971,#101972,#101973,#101974,
#101975,#101976,#101977,#101978,#101979,#101980,#101981,#101982,#101983,
#101984,#101985,#101986,#101987,#101988,#101989,#101990,#101991,#101992,
#101993,#101994,#101995,#101996,#101997,#101998,#101999,#102000,#102001,
#102002,#102003,#102004,#102005,#102006,#102007,#102008,#102009,#102010,
#102011,#102012,#102013,#102014,#102015,#102016,#102017,#102018,#102019,
#102020,#102021,#102022,#102023,#102024,#102025,#102026,#102027,#102028,
#102029,#102030,#102031,#102032,#102033,#102034,#102035,#102036,#102037,
#102038,#102039,#102040,#102041,#102042,#102043,#102044,#102045,#102046,
#102047,#102048,#102049,#102050,#102051,#102052,#102053,#102054,#102055,
#102056,#102057,#102058,#102059,#102060,#102061,#102062,#102063,#102064,
#102065,#102066,#102067,#102068,#102069,#102070,#102071,#102072,#102073,
#102074,#102075,#102076,#102077,#102078,#102079,#102080,#102081,#102082,
#102083,#102084,#102085,#102086,#102087),.UNSPECIFIED.,.F.,.F.,(4,3,3,3,
3,3,3,3,3,3,3,3,3,3,3,3,3,3,3,3,3,3,3,3,3,3,3,3,3,3,3,3,3,3,3,3,3,3,3,3,
3,3,3,3,3,3,3,3,3,3,3,3,3,3,3,3,3,3,3,3,4),(145.822598481187,145.830121694434,
145.93351643147,146.036757713573,146.139877678953,146.24293224715,146.345955455495,
146.448981298156,146.552114064923,146.655303156321,146.758675149692,146.828958144396,
146.932352881429,147.03559416353,147.138714128907,147.241768697101,147.344791905443,
147.4478177481,147.550950514863,147.654139606258,147.757511599624,147.827794594357,
147.931189331481,148.034430613672,148.13755057914,148.240605147424,148.343628355858,
148.446654198605,148.549786965458,148.652976056941,148.756348050395,148.826631044319,
148.930025781262,149.033267063273,149.136387028562,149.239441596668,149.342464804924,
149.445490647496,149.548623414175,149.651812505487,149.755184498774,149.825467494281,
149.928862231266,150.032103513317,150.135223478643,150.238278046785,150.341301255075,
150.444327097678,150.547459864387,150.650648955727,150.754020949038,150.824303944243,
150.927703487101,151.031158736827,151.134277043374,151.23732809389,151.340345927056,
151.444095816518,151.547200209519,151.651272847212,151.755345484905),
 .UNSPECIFIED.);
#1002=B_SPLINE_CURVE_WITH_KNOTS('',3,(#102089,#102090,#102091,#102092,#102093,
#102094,#102095,#102096,#102097,#102098,#102099,#102100,#102101,#102102,
#102103,#102104,#102105,#102106,#102107,#102108,#102109,#102110,#102111,
#102112,#102113,#102114,#102115,#102116,#102117,#102118,#102119,#102120,
#102121,#102122,#102123,#102124,#102125,#102126,#102127,#102128,#102129,
#102130,#102131,#102132,#102133,#102134,#102135,#102136,#102137,#102138,
#102139,#102140,#102141,#102142,#102143,#102144,#102145,#102146,#102147,
#102148,#102149,#102150,#102151,#102152,#102153,#102154,#102155,#102156,
#102157,#102158,#102159,#102160,#102161,#102162,#102163,#102164,#102165,
#102166,#102167,#102168,#102169,#102170,#102171,#102172,#102173,#102174,
#102175,#102176,#102177,#102178,#102179,#102180,#102181,#102182,#102183,
#102184,#102185,#102186,#102187,#102188,#102189,#102190,#102191,#102192,
#102193,#102194,#102195,#102196,#102197,#102198,#102199,#102200,#102201,
#102202,#102203,#102204,#102205,#102206,#102207,#102208,#102209,#102210,
#102211,#102212,#102213,#102214,#102215,#102216,#102217,#102218,#102219,
#102220,#102221,#102222,#102223,#102224,#102225,#102226,#102227,#102228,
#102229,#102230,#102231,#102232,#102233,#102234,#102235,#102236,#102237,
#102238,#102239,#102240,#102241,#102242,#102243,#102244,#102245,#102246,
#102247,#102248,#102249,#102250,#102251,#102252,#102253,#102254,#102255,
#102256,#102257,#102258,#102259,#102260,#102261,#102262,#102263,#102264,
#102265,#102266,#102267,#102268,#102269,#102270,#102271,#102272,#102273,
#102274,#102275,#102276,#102277,#102278,#102279,#102280,#102281,#102282,
#102283,#102284,#102285,#102286,#102287,#102288,#102289,#102290,#102291,
#102292,#102293,#102294,#102295,#102296,#102297,#102298,#102299,#102300,
#102301,#102302,#102303,#102304,#102305,#102306,#102307,#102308,#102309,
#102310,#102311,#102312),.UNSPECIFIED.,.F.,.F.,(4,2,2,2,2,2,2,2,2,2,2,2,
2,2,2,2,2,2,2,2,2,2,2,2,2,2,2,2,2,2,2,2,2,2,2,2,2,2,2,2,2,2,2,2,2,2,2,2,
2,2,2,2,2,2,2,2,2,2,2,2,2,2,2,2,2,2,2,2,2,2,2,2,2,2,2,2,2,2,2,2,2,2,2,2,
2,2,2,2,2,2,2,2,2,2,2,2,2,2,2,2,2,2,2,2,2,2,2,2,2,2,2,4),(-1.25985604642124,
-1.24997270655081,-1.22734490530893,-1.22449277804107,-1.22311614319518,
-1.22204230805192,-1.22080618535122,-1.21862715035613,-1.20881817752338,
-1.15991368846936,-1.12479503245296,-1.12049941387325,-1.11795791125828,
-1.11601698974665,-1.11394341775658,-1.1106943354787,-1.10038219488761,
-1.08381869971055,-1.05095599984349,-1.03712782878735,-1.03047851317781,
-1.01500486154962,-1.01240780738985,-1.01106532121958,-1.00999424463989,
-1.00873359583445,-1.0064418308268,-0.994795494656133,-0.967530279183534,
-0.947345782328875,-0.912838109771735,-0.908551488846451,-0.906012618841815,
-0.904072156114286,-0.901997567960173,-0.898743744060173,-0.888389920536443,
-0.871734055376915,-0.838795169106305,-0.820071561554565,-0.803158463282142,
-0.800503302317016,-0.799148326421416,-0.798076432464727,-0.796825368133199,
-0.794577651366278,-0.783693129837423,-0.759400920475859,-0.703899354149075,
-0.697224257985395,-0.694677030704228,-0.692848931237895,-0.690911210355583,
-0.688344654060897,-0.682716637051382,-0.675223106583611,-0.656363650866931,
-0.626425247443481,-0.604611365836883,-0.590943342810621,-0.588655218165676,
-0.587271113473261,-0.58619417280993,-0.5849776694788,-0.582886707269278,
-0.574276576288882,-0.557513645220457,-0.515491962883698,-0.488621724276845,
-0.484503802915049,-0.482014415016537,-0.480081929702114,-0.477986219744017,
-0.474635587473701,-0.463399237719763,-0.444734219807898,-0.416475451360396,
-0.379486425232132,-0.37664863960059,-0.37527504939945,-0.374201756843105,
-0.372964184162579,-0.37077760542634,-0.361224605495686,-0.312153218603028,
-0.2769866164246,-0.272691422182474,-0.270150399236703,-0.268209975686894,
-0.266137063319112,-0.262889281065477,-0.252778729953164,-0.236574307317366,
-0.198328832770132,-0.167652335690321,-0.16473994695652,-0.163351838579395,
-0.162277199954153,-0.161049276195866,-0.159757267660685,-0.155110071548611,
-0.128864883473422,-0.106990879666121,-0.105559686826295,-0.0651105010710382,
-0.0603738607572403,-0.0579480734197528,-0.0560290631069845,-0.0538783933845104,
-0.0516516908266748,-0.0483298716554019,-0.000628983746475497),
 .UNSPECIFIED.);
#1003=B_SPLINE_CURVE_WITH_KNOTS('',3,(#102313,#102314,#102315,#102316,#102317,
#102318,#102319,#102320,#102321,#102322,#102323,#102324,#102325,#102326,
#102327,#102328,#102329,#102330,#102331,#102332),.UNSPECIFIED.,.F.,.F.,
(4,2,2,2,2,2,2,2,2,4),(-2.6677002844498,-2.62474750340299,-2.62181352290306,
-2.62013078745661,-2.61862587933799,-2.61753430633498,-2.61650703011106,
-2.6147575335521,-2.60998370547245,-2.59357457362298),.UNSPECIFIED.);
#1004=B_SPLINE_CURVE_WITH_KNOTS('',3,(#102337,#102338,#102339,#102340,#102341,
#102342,#102343,#102344,#102345,#102346,#102347,#102348,#102349,#102350,
#102351,#102352,#102353,#102354,#102355,#102356,#102357,#102358,#102359,
#102360,#102361,#102362,#102363,#102364,#102365,#102366,#102367,#102368,
#102369,#102370,#102371,#102372,#102373,#102374,#102375,#102376,#102377,
#102378,#102379,#102380,#102381,#102382,#102383,#102384,#102385,#102386,
#102387,#102388,#102389,#102390,#102391,#102392,#102393,#102394,#102395,
#102396,#102397,#102398,#102399,#102400,#102401,#102402,#102403,#102404,
#102405,#102406,#102407,#102408,#102409,#102410,#102411,#102412,#102413,
#102414,#102415,#102416,#102417,#102418,#102419,#102420,#102421,#102422,
#102423,#102424,#102425,#102426,#102427,#102428,#102429,#102430,#102431,
#102432,#102433,#102434,#102435,#102436,#102437,#102438,#102439,#102440,
#102441,#102442,#102443,#102444,#102445,#102446,#102447,#102448,#102449,
#102450,#102451,#102452,#102453,#102454,#102455,#102456,#102457,#102458,
#102459,#102460,#102461,#102462,#102463,#102464,#102465,#102466,#102467,
#102468,#102469,#102470,#102471,#102472,#102473,#102474,#102475,#102476,
#102477,#102478,#102479,#102480,#102481,#102482,#102483,#102484,#102485,
#102486,#102487,#102488,#102489,#102490,#102491,#102492,#102493,#102494,
#102495,#102496,#102497,#102498,#102499,#102500,#102501,#102502,#102503,
#102504,#102505,#102506,#102507,#102508,#102509,#102510,#102511,#102512,
#102513,#102514,#102515,#102516,#102517,#102518,#102519,#102520,#102521,
#102522,#102523,#102524,#102525,#102526,#102527,#102528,#102529,#102530,
#102531,#102532,#102533,#102534,#102535,#102536,#102537,#102538,#102539,
#102540,#102541,#102542,#102543,#102544,#102545,#102546,#102547,#102548,
#102549,#102550,#102551,#102552,#102553,#102554,#102555,#102556,#102557,
#102558,#102559,#102560,#102561,#102562,#102563,#102564,#102565,#102566,
#102567,#102568,#102569,#102570,#102571,#102572,#102573,#102574,#102575,
#102576,#102577,#102578,#102579,#102580,#102581,#102582,#102583,#102584,
#102585,#102586,#102587,#102588,#102589,#102590,#102591,#102592,#102593,
#102594,#102595,#102596,#102597,#102598,#102599,#102600,#102601,#102602,
#102603,#102604,#102605,#102606,#102607,#102608,#102609,#102610,#102611,
#102612),.UNSPECIFIED.,.F.,.F.,(4,2,2,2,2,2,2,2,2,2,2,2,2,2,2,2,2,2,2,2,
2,2,2,2,2,2,2,2,2,2,2,2,2,2,2,2,2,2,2,2,2,2,2,2,2,2,2,2,2,2,2,2,2,2,2,2,
2,2,2,2,2,2,2,2,2,2,2,2,2,2,2,2,2,2,2,2,2,2,2,2,2,2,2,2,2,2,2,2,2,2,2,2,
2,2,2,2,2,2,2,2,2,2,2,2,2,2,2,2,2,2,2,2,2,2,2,2,2,2,2,2,2,2,2,2,2,2,2,2,
2,2,2,2,2,2,2,2,2,4),(-1.40847138255639,-1.3930392354306,-1.38269162152927,
-1.37943872755714,-1.37736449411351,-1.3754241966515,-1.3728853042098,-1.36859814330709,
-1.33401722799158,-1.27805194810483,-1.27377815670641,-1.27210659414637,
-1.27109457352481,-1.26999224662054,-1.26842734028213,-1.2645148479626,
-1.24530270466621,-1.18892923953642,-1.17208436580389,-1.16846769201748,
-1.16610361687919,-1.16418983950316,-1.16199770675431,-1.15821144155428,
-1.14196490929422,-1.08449072479498,-1.07951866327211,-1.06353363353854,
-1.06091531845003,-1.05956827875815,-1.0584969630881,-1.05723997029619,
-1.05496490110614,-1.04361367011582,-1.01753130893937,-0.964662362292203,
-0.957759473819122,-0.954891474404148,-0.953098290661852,-0.951137059094502,
-0.94843098289729,-0.942012878206311,-0.913438963293679,-0.862245329411575,
-0.851082848859158,-0.848929609514312,-0.84757123893153,-0.846499133412448,
-0.845250662768653,-0.843014678589856,-0.832321719669709,-0.808736040477737,
-0.752159285249997,-0.745595564561645,-0.743065980024229,-0.741242591967052,
-0.739302522367586,-0.736720317983567,-0.731006604842131,-0.708001687506784,
-0.67497997360631,-0.653842589358095,-0.639425012080224,-0.63710057987157,
-0.635705828219258,-0.634627565781027,-0.633417354671249,-0.631354592976211,
-0.623094255513504,-0.607342371482614,-0.565289505582135,-0.537102827248444,
-0.53295100083903,-0.530451711676749,-0.528517807623457,-0.526426802432169,
-0.523097188102357,-0.512056781766311,-0.493846527510116,-0.444761314335446,
-0.427658145115539,-0.42499619947284,-0.423639888499567,-0.422568039156383,
-0.421318292717594,-0.419076103659263,-0.408279038403085,-0.384309248695111,
-0.328332193337035,-0.321706535653096,-0.319167258421557,-0.317341433266562,
-0.315402965105603,-0.312830046862806,-0.307166203583433,-0.284529959069611,
-0.233320767504336,-0.231007914950522,-0.215553274769492,-0.212979023141689,
-0.211656295505932,-0.210636796956037,-0.210628818843005,-0.210621007703407,
-0.210613353319925,-0.210605846222377,-0.210598477624496,-0.210591239463591,
-0.210584124151352,-0.210577124630462,-0.210570234359993,-0.210563447155905,
-0.210556757387543,-0.210550159574956,-0.210543648645456,-0.210537219814358,
-0.210530868647234,-0.210524590888147,-0.210518382518939,-0.21051223973231,
-0.210506158877642,-0.210500136579285,-0.210494169547824,-0.210488254601243,
-0.210482388855394,-0.210476569495251,-0.209213076515601,-0.206823862893776,
-0.193227817559046,-0.156857914973535,-0.113405658750385,-0.109106791554842,
-0.106564686649097,-0.104624064738684,-0.102551548875404,-0.0993056573426866,
-0.0890165731811178,-0.0749180422499143),.UNSPECIFIED.);
#1005=B_SPLINE_CURVE_WITH_KNOTS('',3,(#102613,#102614,#102615,#102616,#102617,
#102618,#102619,#102620,#102621,#102622,#102623,#102624,#102625,#102626,
#102627,#102628,#102629,#102630,#102631,#102632,#102633,#102634,#102635,
#102636,#102637,#102638,#102639,#102640,#102641,#102642,#102643,#102644,
#102645,#102646,#102647,#102648,#102649,#102650,#102651,#102652,#102653,
#102654,#102655,#102656,#102657,#102658,#102659,#102660,#102661,#102662,
#102663,#102664,#102665,#102666,#102667,#102668,#102669,#102670,#102671,
#102672,#102673,#102674,#102675,#102676,#102677,#102678,#102679,#102680,
#102681,#102682,#102683,#102684,#102685,#102686,#102687,#102688,#102689,
#102690,#102691,#102692,#102693,#102694,#102695,#102696,#102697,#102698,
#102699,#102700,#102701,#102702,#102703,#102704,#102705,#102706,#102707,
#102708,#102709,#102710,#102711,#102712,#102713,#102714,#102715,#102716,
#102717,#102718,#102719,#102720,#102721,#102722,#102723,#102724,#102725,
#102726,#102727,#102728,#102729,#102730,#102731,#102732,#102733,#102734,
#102735,#102736,#102737,#102738,#102739,#102740,#102741,#102742,#102743,
#102744,#102745,#102746,#102747,#102748,#102749,#102750,#102751,#102752,
#102753,#102754,#102755,#102756,#102757,#102758,#102759,#102760,#102761,
#102762,#102763,#102764,#102765,#102766,#102767,#102768,#102769,#102770,
#102771,#102772,#102773,#102774,#102775,#102776,#102777,#102778,#102779,
#102780,#102781,#102782,#102783,#102784,#102785,#102786,#102787,#102788,
#102789,#102790,#102791,#102792,#102793,#102794,#102795,#102796,#102797,
#102798,#102799,#102800,#102801,#102802,#102803,#102804,#102805,#102806,
#102807,#102808,#102809,#102810,#102811,#102812,#102813,#102814,#102815,
#102816,#102817,#102818,#102819,#102820,#102821,#102822,#102823,#102824,
#102825,#102826,#102827,#102828,#102829,#102830,#102831,#102832,#102833,
#102834,#102835,#102836,#102837,#102838,#102839,#102840),.UNSPECIFIED.,
 .F.,.F.,(4,2,2,2,2,2,2,2,2,2,2,2,2,2,2,2,2,2,2,2,2,2,2,2,2,2,2,2,2,2,2,
2,2,2,2,2,2,2,2,2,2,2,2,2,2,2,2,2,2,2,2,2,2,2,2,2,2,2,2,2,2,2,2,2,2,2,2,
2,2,2,2,2,2,2,2,2,2,2,2,2,2,2,2,2,2,2,2,2,2,2,2,2,2,2,2,2,2,2,2,2,2,2,2,
2,2,2,2,2,2,2,2,2,2,4),(-2.59357457362298,-2.5725246031732,-2.55108357278968,
-2.52264233424065,-2.51626160565957,-2.51414626091878,-2.51207239908537,
-2.51013131644929,-2.50758976302121,-2.50329444958505,-2.46820949710224,
-2.41939638744359,-2.40952117414475,-2.40734679825542,-2.40610186369359,
-2.40502908379588,-2.40366506071883,-2.40096818234118,-2.38289149380774,
-2.33711789462775,-2.31735499662168,-2.30961736939984,-2.30390362642351,
-2.30128802836053,-2.29934215798713,-2.29752723212433,-2.29503131691526,
-2.28867505872206,-2.23036968426413,-2.20788111560483,-2.19749175063449,
-2.19527434870366,-2.19402972237077,-2.19295684636823,-2.19159223367025,
-2.1888927643583,-2.17074051284007,-2.12635217434615,-2.09546751996204,
-2.09101781286388,-2.08868261759104,-2.08677008134936,-2.0845546117778,
-2.08076512433499,-2.06614985948285,-2.05388708605766,-2.01348397067698,
-1.99463744705181,-1.98534080099832,-1.98319761890393,-1.98196933060854,
-1.98089419047167,-1.97950518273758,-1.97659003645882,-1.94661749989325,
-1.91158573276047,-1.89278798695755,-1.8814950007506,-1.87813765604313,
-1.87604001256748,-1.8741072788546,-1.87161971118434,-1.86750944454131,
-1.84097071500416,-1.79878882558391,-1.78190106720167,-1.77324686313445,
-1.77115200608305,-1.76993439716414,-1.76885726327654,-1.76747390897173,
-1.76518907996402,-1.75160019849135,-1.74979237495307,-1.70242001914626,
-1.67144482065021,-1.66699281031225,-1.66465718644672,-1.66274469493789,
-1.66052972235876,-1.6567421719414,-1.64214768221655,-1.62988213039964,
-1.58947099502746,-1.57061723898786,-1.56131841981834,-1.55917513564019,
-1.55794685311495,-1.55687175996042,-1.55548286826937,-1.55256816094469,
-1.52373078255813,-1.48561968446398,-1.46809409066987,-1.45735297591777,
-1.4540553000815,-1.45197088747224,-1.4500338026562,-1.44751726833858,-1.44330800783644,
-1.41283336595372,-1.36760785399605,-1.35571528989521,-1.35118019824941,
-1.34787178707464,-1.34640930316602,-1.3453245994328,-1.34413571039383,
-1.34216976275827,-1.33576465163016,-1.33420874407463,-1.31962219983047,
-1.26058066063075,-1.25976514203483),.UNSPECIFIED.);
#1006=B_SPLINE_CURVE_WITH_KNOTS('',3,(#102846,#102847,#102848,#102849,#102850,
#102851,#102852,#102853),.UNSPECIFIED.,.F.,.F.,(4,2,2,4),(-0.0748567535247674,
-0.0732687614006028,-0.0499764445815352,-0.00062947833174663),
 .UNSPECIFIED.);
#1007=B_SPLINE_CURVE_WITH_KNOTS('',3,(#102854,#102855,#102856,#102857,#102858,
#102859,#102860,#102861,#102862,#102863,#102864,#102865,#102866,#102867,
#102868,#102869,#102870,#102871,#102872,#102873,#102874,#102875,#102876,
#102877,#102878,#102879,#102880,#102881,#102882,#102883,#102884,#102885,
#102886,#102887,#102888,#102889,#102890,#102891,#102892,#102893,#102894,
#102895,#102896,#102897,#102898,#102899,#102900,#102901,#102902,#102903,
#102904,#102905,#102906,#102907,#102908,#102909,#102910,#102911,#102912,
#102913,#102914,#102915,#102916,#102917,#102918,#102919,#102920,#102921,
#102922,#102923,#102924,#102925,#102926,#102927,#102928,#102929,#102930,
#102931,#102932,#102933,#102934,#102935,#102936,#102937,#102938,#102939,
#102940,#102941,#102942,#102943,#102944,#102945,#102946,#102947,#102948,
#102949,#102950,#102951,#102952,#102953,#102954,#102955,#102956,#102957,
#102958,#102959,#102960,#102961,#102962,#102963,#102964,#102965,#102966,
#102967,#102968,#102969,#102970,#102971,#102972,#102973,#102974,#102975,
#102976,#102977,#102978,#102979,#102980,#102981,#102982,#102983,#102984,
#102985,#102986,#102987,#102988,#102989,#102990,#102991,#102992,#102993,
#102994,#102995,#102996,#102997,#102998,#102999,#103000,#103001,#103002,
#103003,#103004,#103005,#103006,#103007,#103008,#103009,#103010,#103011,
#103012,#103013,#103014,#103015,#103016,#103017,#103018,#103019,#103020,
#103021,#103022,#103023,#103024,#103025,#103026,#103027,#103028,#103029,
#103030,#103031,#103032,#103033,#103034,#103035,#103036,#103037,#103038,
#103039,#103040,#103041,#103042,#103043,#103044,#103045,#103046,#103047,
#103048,#103049,#103050,#103051,#103052,#103053,#103054,#103055,#103056,
#103057,#103058,#103059,#103060,#103061,#103062,#103063,#103064,#103065,
#103066,#103067,#103068,#103069,#103070,#103071,#103072,#103073,#103074,
#103075,#103076,#103077,#103078,#103079,#103080,#103081,#103082,#103083,
#103084,#103085,#103086,#103087,#103088,#103089,#103090,#103091,#103092,
#103093,#103094,#103095,#103096,#103097,#103098,#103099,#103100,#103101,
#103102,#103103,#103104,#103105,#103106,#103107,#103108,#103109,#103110,
#103111),.UNSPECIFIED.,.F.,.F.,(4,2,2,2,2,2,2,2,2,2,2,2,2,2,2,2,2,2,2,2,
2,2,2,2,2,2,2,2,2,2,2,2,2,2,2,2,2,2,2,2,2,2,2,2,2,2,2,2,2,2,2,2,2,2,2,2,
2,2,2,2,2,2,2,2,2,2,2,2,2,2,2,2,2,2,2,2,2,2,2,2,2,2,2,2,2,2,2,2,2,2,2,2,
2,2,2,2,2,2,2,2,2,2,2,2,2,2,2,2,2,2,2,2,2,2,2,2,2,2,2,2,2,2,2,2,2,2,2,2,
4),(-2.66781222492019,-2.66001838762793,-2.6547219431894,-2.65227856128054,
-2.65039670419209,-2.64855599431708,-2.64672958842394,-2.64418919325558,
-2.63899802022748,-2.62648778430856,-2.57481848753383,-2.55597610161522,
-2.54668119359671,-2.54453832547705,-2.5433102031511,-2.54223519917316,
-2.54084635531448,-2.53793151047647,-2.50823512364153,-2.45778623830298,
-2.44829727953654,-2.44369003448626,-2.43991096150434,-2.43774027301652,
-2.43772457867808,-2.43770833179418,-2.43769151228051,-2.43767409920081,
-2.43765607096917,-2.43763740524581,-2.43761807882281,-2.43759806759226,
-2.43757734664654,-2.43755589023898,-2.43753367159252,-2.43751066235144,
-2.43749062627382,-2.43746727622944,-2.43744007012691,-2.4374083799564,
-2.43737147940545,-2.43732853023764,-2.43727431906842,-2.43533361120814,
-2.43279161819176,-2.42849347585957,-2.39337252264298,-2.34441469832562,
-2.33471462311872,-2.33254340900183,-2.33130917572928,-2.33023535387445,
-2.32885659612426,-2.32599271201286,-2.29003732511163,-2.25727199776668,
-2.23471252911173,-2.22905913989001,-2.22648797558917,-2.22454961251538,
-2.22272299680303,-2.22018119330167,-2.21354042279847,-2.15773544341966,
-2.13367372059929,-2.12285065304746,-2.1206067486876,-2.11935654883769,
-2.11828462458865,-2.11692861431965,-2.11478310271424,-2.10374657939899,
-2.05252997599714,-2.02382110510827,-2.01738747719566,-2.01467883356504,
-2.01271718730132,-2.01092462299219,-2.00805977523021,-2.00117563801035,
-1.94810072624431,-1.92219395636758,-1.9108869405113,-1.90861449989724,
-1.90735810663759,-1.90628678781813,-1.90493908338821,-1.90231753500915,
-1.88627571696096,-1.88098515593715,-1.86640073972647,-1.83350915867338,
-1.81694245916113,-1.80663015251884,-1.80338122656909,-1.80130781087837,
-1.79936707591627,-1.79682587686432,-1.79253093632626,-1.7574192793556,
-1.70851520795402,-1.69874469197343,-1.69656848733368,-1.6953330785133,
-1.69425929790861,-1.69288198420773,-1.69002589122103,-1.66722643173411,
-1.61161804068732,-1.59560669677266,-1.59183726382131,-1.58964881155249,
-1.58773462514935,-1.58536536578613,-1.58173203162915,-1.56463510149431,
-1.55656647867173,-1.52175631463101,-1.49770679491481,-1.486887272655,-1.48464367581751,
-1.4833935873754,-1.48232172169696,-1.48096573811559,-1.47830548185271,
-1.46125216265378,-1.44264026103571,-1.40968433184212,-1.40847138255639),
 .UNSPECIFIED.);
#1008=B_SPLINE_CURVE_WITH_KNOTS('',3,(#103113,#103114,#103115,#103116,#103117,
#103118,#103119,#103120,#103121,#103122,#103123,#103124,#103125,#103126,
#103127,#103128,#103129,#103130,#103131,#103132,#103133,#103134,#103135,
#103136,#103137,#103138,#103139,#103140,#103141,#103142,#103143,#103144,
#103145,#103146,#103147,#103148,#103149,#103150,#103151,#103152,#103153,
#103154,#103155,#103156,#103157,#103158,#103159,#103160,#103161,#103162,
#103163,#103164,#103165,#103166,#103167,#103168,#103169,#103170,#103171,
#103172,#103173,#103174,#103175,#103176,#103177,#103178,#103179,#103180,
#103181,#103182,#103183,#103184,#103185,#103186,#103187,#103188,#103189,
#103190,#103191,#103192,#103193,#103194,#103195,#103196,#103197,#103198,
#103199,#103200,#103201,#103202,#103203,#103204,#103205,#103206,#103207,
#103208,#103209,#103210,#103211,#103212,#103213,#103214,#103215,#103216,
#103217,#103218,#103219,#103220,#103221,#103222,#103223,#103224,#103225,
#103226,#103227,#103228,#103229,#103230,#103231,#103232,#103233,#103234,
#103235,#103236,#103237,#103238,#103239,#103240,#103241,#103242,#103243,
#103244,#103245,#103246,#103247,#103248,#103249,#103250,#103251,#103252,
#103253,#103254,#103255,#103256,#103257,#103258,#103259,#103260,#103261,
#103262,#103263,#103264,#103265,#103266,#103267,#103268,#103269,#103270,
#103271,#103272,#103273,#103274,#103275,#103276,#103277,#103278,#103279,
#103280,#103281,#103282,#103283,#103284,#103285,#103286,#103287,#103288,
#103289,#103290,#103291,#103292,#103293,#103294,#103295,#103296,#103297,
#103298,#103299,#103300,#103301,#103302,#103303,#103304,#103305,#103306,
#103307,#103308,#103309,#103310,#103311,#103312,#103313,#103314,#103315,
#103316,#103317,#103318,#103319,#103320,#103321,#103322),.UNSPECIFIED.,
 .F.,.F.,(4,2,2,2,2,2,2,2,2,2,2,2,2,2,2,2,2,2,2,2,2,2,2,2,2,2,2,2,2,2,2,
2,2,2,2,2,2,2,2,2,2,2,2,2,2,2,2,2,2,2,2,2,2,2,2,2,2,2,2,2,2,2,2,2,2,2,2,
2,2,2,2,2,2,2,2,2,2,2,2,2,2,2,2,2,2,2,2,2,2,2,2,2,2,2,2,2,2,2,2,2,2,2,2,
2,4),(-1.25976514203483,-1.24627096371811,-1.24250927652393,-1.24030044353385,
-1.23838778851667,-1.23604506193199,-1.2315581355053,-1.19919642732524,
-1.15901287546397,-1.154080862944,-1.13813164183323,-1.13551512195141,-1.13416841297433,
-1.1330970481481,-1.13183963557149,-1.12956288498489,-1.11818426966118,
-1.09199516951617,-1.03927233402488,-1.03235781358755,-1.02948777677141,
-1.02769413151857,-1.02573304724538,-1.0230283682676,-1.01661921625226,
-0.988122027355997,-0.937199033953814,-0.92570732222101,-0.923534283368015,
-0.92216983946654,-0.921097179097549,-0.919852904953113,-0.917636368444082,
-0.907255775161229,-0.884792459204342,-0.826429150771745,-0.820076724627021,
-0.817581759295738,-0.815767332801416,-0.813821817771153,-0.811206375776999,
-0.805309368346198,-0.780917436221713,-0.730252743974468,-0.714075036808931,
-0.71144853251101,-0.710099726687497,-0.709028290787664,-0.70777264416632,
-0.705503785067525,-0.694260549833938,-0.668601107664333,-0.615122712521193,
-0.608267228794461,-0.605407019377386,-0.603615243533792,-0.601652763109141,
-0.598939841635263,-0.592481172117712,-0.538597461479476,-0.502336141671931,
-0.499483271458002,-0.498106611474066,-0.497032913624168,-0.495797126220781,
-0.493619106870349,-0.483821762615518,-0.434915951358219,-0.399786429157354,
-0.395498805114655,-0.392959812225597,-0.39101952733057,-0.388945393145167,
-0.385692833110238,-0.375347705471159,-0.358710291130442,-0.325789163427632,
-0.307660674855151,-0.290153697049808,-0.287477078436241,-0.286117619946777,
-0.285045511777135,-0.283798019624447,-0.281566221948021,-0.2709389051044,
-0.247590817162665,-0.191922910262866,-0.184490884349839,-0.181533970338131,
-0.179724538613804,-0.177895292514631,-0.175385725401274,-0.170037645275231,
-0.162927961360404,-0.145450036545872,-0.0958298182879772,-0.0781715427825538,
-0.0754897006043806,-0.0741291637744639,-0.0730570135908618,-0.0718103986139602,
-0.0695824611675837,-0.0590160995158885,-0.0358876316419884,-0.000629543614865904),
 .UNSPECIFIED.);
#1009=B_SPLINE_CURVE_WITH_KNOTS('',3,(#103323,#103324,#103325,#103326,#103327,
#103328,#103329,#103330,#103331,#103332,#103333,#103334,#103335,#103336,
#103337,#103338,#103339,#103340,#103341,#103342,#103343,#103344),
 .UNSPECIFIED.,.F.,.F.,(4,2,2,2,2,2,2,2,2,2,4),(-2.66754968025911,-2.64222557872969,
-2.63909886152637,-2.6369529653842,-2.63515231182392,-2.6332385260983,-2.63086956528686,
-2.62723631926054,-2.6101324181504,-2.59794289122828,-2.59313490574478),
 .UNSPECIFIED.);
#1010=B_SPLINE_CURVE_WITH_KNOTS('',3,(#103349,#103350,#103351,#103352,#103353,
#103354,#103355,#103356,#103357,#103358,#103359,#103360,#103361,#103362,
#103363,#103364,#103365,#103366,#103367,#103368,#103369,#103370,#103371,
#103372,#103373,#103374,#103375,#103376,#103377,#103378,#103379,#103380,
#103381,#103382,#103383,#103384,#103385,#103386,#103387,#103388,#103389,
#103390,#103391,#103392,#103393,#103394,#103395,#103396,#103397,#103398,
#103399,#103400,#103401,#103402,#103403,#103404,#103405,#103406,#103407,
#103408,#103409,#103410,#103411,#103412,#103413,#103414,#103415,#103416,
#103417,#103418,#103419,#103420,#103421,#103422,#103423,#103424,#103425,
#103426,#103427,#103428,#103429,#103430,#103431,#103432,#103433,#103434,
#103435,#103436,#103437,#103438,#103439,#103440,#103441,#103442,#103443,
#103444,#103445,#103446,#103447,#103448,#103449,#103450,#103451,#103452,
#103453,#103454,#103455,#103456,#103457,#103458,#103459,#103460,#103461,
#103462,#103463,#103464,#103465,#103466,#103467,#103468,#103469,#103470,
#103471,#103472,#103473,#103474,#103475,#103476,#103477,#103478,#103479,
#103480,#103481,#103482,#103483,#103484,#103485,#103486,#103487,#103488,
#103489,#103490,#103491,#103492,#103493,#103494,#103495,#103496,#103497,
#103498,#103499,#103500,#103501,#103502,#103503,#103504,#103505,#103506,
#103507,#103508,#103509,#103510,#103511,#103512,#103513,#103514,#103515,
#103516,#103517,#103518,#103519,#103520,#103521,#103522,#103523,#103524,
#103525,#103526,#103527,#103528,#103529,#103530,#103531,#103532,#103533,
#103534,#103535,#103536,#103537,#103538,#103539,#103540,#103541,#103542,
#103543,#103544,#103545,#103546,#103547,#103548,#103549,#103550,#103551,
#103552,#103553,#103554,#103555,#103556,#103557,#103558,#103559,#103560,
#103561,#103562,#103563,#103564,#103565,#103566,#103567,#103568,#103569,
#103570,#103571,#103572,#103573,#103574,#103575,#103576,#103577,#103578,
#103579,#103580,#103581,#103582,#103583,#103584,#103585,#103586,#103587,
#103588,#103589,#103590),.UNSPECIFIED.,.F.,.F.,(4,2,2,2,2,2,2,2,2,2,2,2,
2,2,2,2,2,2,2,2,2,2,2,2,2,2,2,2,2,2,2,2,2,2,2,2,2,2,2,2,2,2,2,2,2,2,2,2,
2,2,2,2,2,2,2,2,2,2,2,2,2,2,2,2,2,2,2,2,2,2,2,2,2,2,2,2,2,2,2,2,2,2,2,2,
2,2,2,2,2,2,2,2,2,2,2,2,2,2,2,2,2,2,2,2,2,2,2,2,2,2,2,2,2,2,2,2,2,2,2,2,
4),(-1.40835436178516,-1.40120748467684,-1.37505305271072,-1.36368250096922,
-1.36140621418413,-1.36014888904888,-1.35907749999195,-1.35773062880308,
-1.35511340876948,-1.33915136590534,-1.33420734953041,-1.32856139629404,
-1.28160143233727,-1.28015780613655,-1.26111694966373,-1.25735565670909,
-1.25494685966479,-1.25302909761683,-1.25086691763213,-1.24721719786922,
-1.2327660419842,-1.1823778016643,-1.15270966940492,-1.14979517135514,-1.14840640334139,
-1.14733141310644,-1.14610326547807,-1.14396024280758,-1.13466326363675,
-1.11581174254254,-1.07535841393395,-1.06307969665175,-1.04849987361659,
-1.0447138919679,-1.0424994337114,-1.04058714143595,-1.03825145285354,-1.03379836669918,
-1.00276226937868,-0.954784645856903,-0.940195549477655,-0.937863185595314,
-0.936465945171996,-0.935387147829541,-0.934177885721391,-0.932120170614113,
-0.923924762041621,-0.908358607240402,-0.866775225235952,-0.854638989158886,
-0.836943366883324,-0.833270679930094,-0.830889086290468,-0.82897367800387,
-0.826793330569765,-0.823061595502939,-0.807565125555238,-0.755635584891186,
-0.728680061603705,-0.725778524655203,-0.724392241475761,-0.723317470188229,
-0.722087662996888,-0.719937259692629,-0.710538472974241,-0.661283210068209,
-0.626056494999795,-0.621759540475693,-0.619217674914547,-0.617276722352837,
-0.615203355791732,-0.611955093503761,-0.601649752815576,-0.585101169720129,
-0.552251199323677,-0.539685406155158,-0.516623260530808,-0.513766768776718,
-0.512389378818381,-0.511315589921085,-0.510080237757896,-0.50790427768254,
-0.498137604845868,-0.449204626363468,-0.414080325033906,-0.409784352877915,
-0.407242910031934,-0.405302189042837,-0.403228981430708,-0.399980783576168,
-0.389674092098935,-0.373121861408414,-0.340270899400875,-0.327215628598037,
-0.318559273272307,-0.304219898924665,-0.301897168864333,-0.300502890290625,
-0.29942465718587,-0.298214103100781,-0.296149922239845,-0.287872932045477,
-0.272073958306711,-0.226218489024688,-0.201664173317549,-0.197636537294232,
-0.195173837035319,-0.193301738838713,-0.191274958300659,-0.188089451327945,
-0.184342526667239,-0.177228317181495,-0.159734752796449,-0.110014209964816,
-0.0924687521570684,-0.0897907578290559,-0.0884310004100348,-0.0873588619835297,
-0.0861115701772213,-0.0838807143168502,-0.0748567535247674),
 .UNSPECIFIED.);
#1011=B_SPLINE_CURVE_WITH_KNOTS('',3,(#103591,#103592,#103593,#103594,#103595,
#103596,#103597,#103598,#103599,#103600,#103601,#103602,#103603,#103604,
#103605,#103606,#103607,#103608,#103609,#103610,#103611,#103612,#103613,
#103614,#103615,#103616,#103617,#103618,#103619,#103620,#103621,#103622,
#103623,#103624,#103625,#103626,#103627,#103628,#103629,#103630,#103631,
#103632,#103633,#103634,#103635,#103636,#103637,#103638,#103639,#103640,
#103641,#103642,#103643,#103644,#103645,#103646,#103647,#103648,#103649,
#103650,#103651,#103652,#103653,#103654,#103655,#103656,#103657,#103658,
#103659,#103660,#103661,#103662,#103663,#103664,#103665,#103666,#103667,
#103668,#103669,#103670,#103671,#103672,#103673,#103674,#103675,#103676,
#103677,#103678,#103679,#103680,#103681,#103682,#103683,#103684,#103685,
#103686,#103687,#103688,#103689,#103690,#103691,#103692,#103693,#103694,
#103695,#103696,#103697,#103698,#103699,#103700,#103701,#103702,#103703,
#103704,#103705,#103706,#103707,#103708,#103709,#103710,#103711,#103712,
#103713,#103714,#103715,#103716,#103717,#103718,#103719,#103720,#103721,
#103722,#103723,#103724,#103725,#103726,#103727,#103728,#103729,#103730,
#103731,#103732,#103733,#103734,#103735,#103736,#103737,#103738,#103739,
#103740,#103741,#103742,#103743,#103744,#103745,#103746,#103747,#103748,
#103749,#103750,#103751,#103752,#103753,#103754,#103755,#103756,#103757,
#103758,#103759,#103760,#103761,#103762,#103763,#103764,#103765,#103766,
#103767,#103768,#103769,#103770,#103771,#103772,#103773,#103774,#103775,
#103776,#103777,#103778,#103779,#103780,#103781,#103782,#103783,#103784,
#103785,#103786,#103787,#103788,#103789,#103790,#103791,#103792,#103793,
#103794,#103795,#103796,#103797,#103798,#103799,#103800,#103801,#103802,
#103803,#103804,#103805,#103806,#103807,#103808,#103809,#103810,#103811,
#103812,#103813,#103814,#103815,#103816,#103817,#103818,#103819,#103820,
#103821,#103822,#103823,#103824,#103825,#103826,#103827,#103828,#103829,
#103830,#103831,#103832,#103833,#103834,#103835,#103836,#103837,#103838,
#103839,#103840,#103841,#103842,#103843,#103844,#103845,#103846,#103847,
#103848,#103849,#103850,#103851,#103852,#103853,#103854,#103855,#103856,
#103857,#103858,#103859,#103860,#103861,#103862,#103863,#103864,#103865,
#103866),.UNSPECIFIED.,.F.,.F.,(4,2,2,2,2,2,2,2,2,2,2,2,2,2,2,2,2,2,2,2,
2,2,2,2,2,2,2,2,2,2,2,2,2,2,2,2,2,2,2,2,2,2,2,2,2,2,2,2,2,2,2,2,2,2,2,2,
2,2,2,2,2,2,2,2,2,2,2,2,2,2,2,2,2,2,2,2,2,2,2,2,2,2,2,2,2,2,2,2,2,2,2,2,
2,2,2,2,2,2,2,2,2,2,2,2,2,2,2,2,2,2,2,2,2,2,2,2,2,2,2,2,2,2,2,2,2,2,2,2,
2,2,2,2,2,2,2,2,2,4),(-2.59313490574478,-2.55330326801384,-2.53483436151909,
-2.5310022515763,-2.52945059810669,-2.52835100895761,-2.5273363692964,-2.52565012427039,
-2.5212842676782,-2.47357798675594,-2.44429013327263,-2.43427814598053,
-2.42949034686026,-2.42559713121777,-2.42339376444406,-2.4233810955763,
-2.42336798932302,-2.42335442953436,-2.42334039932334,-2.42332587818603,
-2.42331084945732,-2.42329529574739,-2.42327919728274,-2.42326253346499,
-2.42324528285917,-2.42322742314613,-2.4232089310934,-2.42318978253747,
-2.42316995227465,-2.42314941408245,-2.42312814067539,-2.42310610361413,
-2.42308327274177,-2.4230639674276,-2.42304141425639,-2.42301506360632,
-2.42298427229399,-2.4229482878032,-2.42290622989389,-2.42285835310031,
-2.42091785871573,-2.41837621358731,-2.41407881259393,-2.37897334829359,
-2.33005825774277,-2.32031470827636,-2.31814066016904,-2.31690588134865,
-2.31583226771662,-2.31445467047015,-2.3115962759417,-2.28868622423929,
-2.24625632528545,-2.22764346886388,-2.21643091968091,-2.21308300383397,
-2.21098802371109,-2.20905555419177,-2.20656527006203,-2.20244391464848,
-2.17517766963749,-2.13299297660313,-2.11667461410578,-2.10821630695699,
-2.10613757097069,-2.10492385879532,-2.10384647192153,-2.10245800952345,
-2.10015481594809,-2.08617274881369,-2.06460740532472,-2.03153810979631,
-2.00850110350888,-2.00278363856421,-2.00020085510439,-1.99826080213208,
-1.99643776369501,-1.99390919727569,-1.98735113380447,-1.93076194716973,
-1.92829418114678,-1.90662743707945,-1.89647520864303,-1.89427366515673,
-1.89303278485856,-1.89195989220095,-1.89059104857492,-1.88840315495372,
-1.87670414775936,-1.87292085431342,-1.87268894626612,-1.86582352375722,
-1.85209117875077,-1.81921046424644,-1.80265569122254,-1.79234891954575,
-1.78910073227713,-1.78702754643769,-1.78508685692137,-1.78254547251614,
-1.77824966985943,-1.74305700781315,-1.69388887139729,-1.68442985126656,
-1.68227541001777,-1.68104482881162,-1.67997038184518,-1.67858582312859,
-1.67569248729687,-1.64965970583749,-1.61149463659113,-1.58246829861086,
-1.57807293184966,-1.57574948913394,-1.57383798981261,-1.57161399045446,
-1.56778594831757,-1.55272544856017,-1.50055993324135,-1.48171540162278,
-1.47242008047358,-1.47027730174263,-1.46904926040354,-1.46797434672869,
-1.46658564515949,-1.46367118942575,-1.43362669393912,-1.38228786957019,
-1.36894840986627,-1.36539355974845,-1.36325252177946,-1.36133134399441,
-1.35888814619682,-1.35501380153761,-1.33394078482172,-1.27612802698394,
-1.26116802669047,-1.25973369591908),.UNSPECIFIED.);
#1012=B_SPLINE_CURVE_WITH_KNOTS('',3,(#103872,#103873,#103874,#103875),
 .UNSPECIFIED.,.F.,.F.,(4,4),(120.339865682355,120.689851223097),
 .UNSPECIFIED.);
#1013=B_SPLINE_CURVE_WITH_KNOTS('',3,(#103876,#103877,#103878,#103879,#103880,
#103881,#103882,#103883,#103884,#103885,#103886,#103887,#103888,#103889,
#103890,#103891,#103892,#103893,#103894,#103895,#103896,#103897,#103898,
#103899,#103900,#103901,#103902,#103903,#103904,#103905,#103906,#103907,
#103908,#103909,#103910,#103911,#103912,#103913,#103914,#103915,#103916,
#103917,#103918,#103919,#103920,#103921,#103922,#103923,#103924,#103925,
#103926,#103927,#103928,#103929,#103930,#103931,#103932,#103933,#103934,
#103935,#103936,#103937,#103938,#103939,#103940,#103941,#103942,#103943,
#103944,#103945,#103946,#103947,#103948,#103949,#103950,#103951,#103952,
#103953,#103954,#103955,#103956,#103957,#103958,#103959,#103960,#103961,
#103962,#103963,#103964,#103965,#103966,#103967,#103968,#103969,#103970,
#103971,#103972,#103973,#103974,#103975,#103976,#103977,#103978,#103979,
#103980,#103981,#103982,#103983,#103984,#103985,#103986,#103987,#103988,
#103989,#103990,#103991,#103992,#103993,#103994,#103995,#103996,#103997,
#103998,#103999,#104000,#104001,#104002,#104003,#104004,#104005,#104006,
#104007,#104008,#104009,#104010,#104011,#104012,#104013,#104014,#104015,
#104016,#104017,#104018,#104019,#104020,#104021,#104022,#104023,#104024,
#104025,#104026,#104027,#104028,#104029,#104030,#104031,#104032,#104033,
#104034,#104035,#104036,#104037,#104038,#104039,#104040,#104041,#104042,
#104043,#104044,#104045,#104046,#104047,#104048,#104049,#104050,#104051,
#104052,#104053,#104054,#104055,#104056,#104057,#104058,#104059,#104060,
#104061,#104062,#104063,#104064,#104065,#104066,#104067,#104068,#104069,
#104070,#104071,#104072,#104073,#104074,#104075,#104076,#104077,#104078,
#104079,#104080,#104081,#104082,#104083,#104084,#104085,#104086,#104087,
#104088,#104089,#104090,#104091,#104092,#104093,#104094,#104095,#104096,
#104097,#104098,#104099,#104100,#104101),.UNSPECIFIED.,.F.,.F.,(4,2,2,2,
2,2,2,2,2,2,2,2,2,2,2,2,2,2,2,2,2,2,2,2,2,2,2,2,2,2,2,2,2,2,2,2,2,2,2,2,
2,2,2,2,2,2,2,2,2,2,2,2,2,2,2,2,2,2,2,2,2,2,2,2,2,2,2,2,2,2,2,2,2,2,2,2,
2,2,2,2,2,2,2,2,2,2,2,2,2,2,2,2,2,2,2,2,2,2,2,2,2,2,2,2,2,2,2,2,2,2,2,2,
4),(-2.66740566330074,-2.64317490644518,-2.6360437625599,-2.63425319807585,
-2.63303838589649,-2.63202935526164,-2.63095478054007,-2.62956857342768,
-2.62666658944157,-2.59961424602175,-2.58553293708982,-2.57351180775184,
-2.54173365275992,-2.53137908523418,-2.52812536151031,-2.52605092363122,
-2.5241106625936,-2.52157214574642,-2.51728635270582,-2.4742491908246,-2.4442673431881,
-2.43065638899947,-2.42319719800404,-2.42121047786026,-2.42019242067258,
-2.41912216435068,-2.41779427060571,-2.41574038253585,-2.40608495751117,
-2.35237118375876,-2.32446089926702,-2.31812322367221,-2.31543091159095,
-2.31347226465107,-2.31167633345679,-2.30879273699945,-2.30179452432377,
-2.25037547417588,-2.22330082846914,-2.21170131424476,-2.20941238508367,
-2.20815244410715,-2.20708145943003,-2.20573843689133,-2.20313844977164,
-2.18759175364158,-2.18102885537958,-2.16576374521916,-2.13787313177137,
-2.11898267497714,-2.11148113981519,-2.10584872664639,-2.10328136176684,
-2.10134352073457,-2.09951567304948,-2.09696938430387,-2.09030024854694,
-2.03477063489238,-2.01052540492794,-1.99965279600475,-1.99740583410008,
-1.9961549379745,-1.99508303698877,-1.99372785132462,-1.9910716819442,-1.97413313727524,
-1.92386907190346,-1.90627531601881,-1.89550485253889,-1.89220441116883,
-1.89011969471492,-1.88818332415432,-1.88566913169197,-1.88146689783177,
-1.85126644148712,-1.79974163337377,-1.78775102877288,-1.78544061349278,
-1.78417595451377,-1.78310520348447,-1.78176782989071,-1.77968325112593,
-1.76959123584787,-1.76409915483254,-1.75667234239292,-1.743164826707,-1.71028301970526,
-1.69372929311369,-1.6834227056449,-1.68017432770869,-1.6781009603903,-1.67616005899206,
-1.67361833651232,-1.66932182652777,-1.6341046684402,-1.58485956810295,
-1.57548192421687,-1.57333313068167,-1.57210371676431,-1.57102895166417,
-1.56964222130379,-1.56739549579956,-1.5545624869472,-1.55239653151165,
-1.50511597875543,-1.47659174138898,-1.47017975600638,-1.46747456192548,
-1.46551335433549,-1.46371977252385,-1.46085020964095,-1.45393873571281,
-1.40835436178516),.UNSPECIFIED.);
#1014=B_SPLINE_CURVE_WITH_KNOTS('',3,(#104103,#104104,#104105,#104106,#104107,
#104108,#104109,#104110,#104111,#104112,#104113,#104114,#104115,#104116,
#104117,#104118,#104119,#104120,#104121,#104122,#104123,#104124,#104125,
#104126,#104127,#104128,#104129,#104130,#104131,#104132,#104133,#104134,
#104135,#104136,#104137,#104138,#104139,#104140,#104141,#104142,#104143,
#104144,#104145,#104146,#104147,#104148,#104149,#104150,#104151,#104152,
#104153,#104154,#104155,#104156,#104157,#104158,#104159,#104160,#104161,
#104162,#104163,#104164,#104165,#104166,#104167,#104168,#104169,#104170,
#104171,#104172,#104173,#104174,#104175,#104176,#104177,#104178,#104179,
#104180,#104181,#104182,#104183,#104184,#104185,#104186,#104187,#104188,
#104189,#104190,#104191,#104192,#104193,#104194,#104195,#104196,#104197,
#104198,#104199,#104200,#104201,#104202,#104203,#104204,#104205,#104206,
#104207,#104208,#104209,#104210,#104211,#104212,#104213,#104214,#104215,
#104216,#104217,#104218,#104219,#104220,#104221,#104222,#104223,#104224,
#104225,#104226,#104227,#104228,#104229,#104230,#104231,#104232,#104233,
#104234,#104235,#104236,#104237,#104238,#104239,#104240,#104241,#104242,
#104243,#104244,#104245,#104246,#104247,#104248,#104249,#104250,#104251,
#104252,#104253,#104254,#104255,#104256,#104257,#104258,#104259,#104260,
#104261,#104262,#104263,#104264,#104265,#104266,#104267,#104268,#104269,
#104270,#104271,#104272,#104273,#104274,#104275,#104276,#104277,#104278,
#104279,#104280,#104281,#104282,#104283,#104284,#104285,#104286,#104287,
#104288,#104289,#104290,#104291,#104292,#104293,#104294,#104295,#104296,
#104297,#104298,#104299,#104300,#104301,#104302,#104303,#104304,#104305,
#104306,#104307,#104308,#104309,#104310,#104311,#104312,#104313,#104314,
#104315,#104316,#104317,#104318,#104319,#104320,#104321,#104322,#104323,
#104324,#104325,#104326),.UNSPECIFIED.,.F.,.F.,(4,2,2,2,2,2,2,2,2,2,2,2,
2,2,2,2,2,2,2,2,2,2,2,2,2,2,2,2,2,2,2,2,2,2,2,2,2,2,2,2,2,2,2,2,2,2,2,2,
2,2,2,2,2,2,2,2,2,2,2,2,2,2,2,2,2,2,2,2,2,2,2,2,2,2,2,2,2,2,2,2,2,2,2,2,
2,2,2,2,2,2,2,2,2,2,2,2,2,2,2,2,2,2,2,2,2,2,2,2,2,2,2,4),(-1.25973369591908,
-1.25882010703106,-1.25741836646077,-1.25633902654265,-1.25513241539184,
-1.25308637675045,-1.245029277895,-1.22985063334681,-1.18995584899926,-1.15891311792271,
-1.1546917298589,-1.15217188560428,-1.1502345426746,-1.14815210177199,-1.14486232251316,
-1.13418906717786,-1.11681833999807,-1.06811645470584,-1.06160140353263,
-1.04897950432908,-1.04674387314019,-1.04536050660888,-1.04428612108112,
-1.04305464910848,-1.04089636336231,-1.03138450553894,-0.982233088275675,
-0.947038879444556,-0.942742708123222,-0.940201192925525,-0.938260442868806,
-0.936187229586887,-0.932939075835942,-0.922632970759417,-0.906082106209736,
-0.87323206225543,-0.860314571933824,-0.837612583026447,-0.834759141645184,
-0.833382428324641,-0.832308793433493,-0.831073196598608,-0.828895795913767,
-0.819105929104722,-0.770197943800586,-0.735082318584062,-0.730787583347391,
-0.728246622193727,-0.726306125035958,-0.724233016917092,-0.720984683435521,
-0.710675104521929,-0.694115899984244,-0.661260969463728,-0.647487449350561,
-0.640719713392962,-0.639092290674091,-0.625191559062593,-0.62289233454933,
-0.62150503156868,-0.620427782873463,-0.619213382334404,-0.617131555436607,
-0.608634898562339,-0.592203006413606,-0.550103306052869,-0.522875939161712,
-0.518749332543588,-0.516257521915162,-0.51432483506572,-0.512230585132612,
-0.508885930337426,-0.497703828023856,-0.479164576426568,-0.43498853085022,
-0.41369061059898,-0.410873471058813,-0.409504015921035,-0.408431166335568,
-0.407190937311453,-0.404991997310929,-0.394877399544114,-0.373335899106141,
-0.363128768521085,-0.314935732240373,-0.307784427807797,-0.304875456329372,
-0.30307499276735,-0.301120321420233,-0.298449562819577,-0.292236469553449,
-0.26534659046944,-0.226490563733547,-0.201853293048104,-0.198976728268952,
-0.197595613296098,-0.19656687565604,-0.195375402799059,-0.193400822351896,
-0.190973660742924,-0.186051016465701,-0.172643559365281,-0.151527626500562,
-0.102990334553856,-0.0958517578786078,-0.0929449766948306,-0.0911449588602478,
-0.0891900531518719,-0.0865176815474027,-0.0802949449086537,-0.0533261439010829,
-0.000629601453589488),.UNSPECIFIED.);
#1015=B_SPLINE_CURVE_WITH_KNOTS('',3,(#104327,#104328,#104329,#104330,#104331,
#104332,#104333,#104334,#104335,#104336,#104337,#104338,#104339,#104340,
#104341,#104342,#104343,#104344,#104345,#104346,#104347,#104348,#104349,
#104350),.UNSPECIFIED.,.F.,.F.,(4,2,2,2,2,2,2,2,2,2,2,4),(-2.66819246569389,
-2.66013468457772,-2.65577695930745,-2.65436379664703,-2.65329641581407,
-2.6522660819304,-2.651086027011,-2.6491605796328,-2.64309431029485,-2.64181214569972,
-2.63401080610002,-2.59392646598523),.UNSPECIFIED.);
#1016=B_SPLINE_CURVE_WITH_KNOTS('',3,(#104356,#104357,#104358,#104359,#104360,
#104361,#104362,#104363,#104364,#104365,#104366,#104367,#104368),
 .UNSPECIFIED.,.F.,.F.,(4,3,3,3,4),(114.057240443604,114.163813834894,114.270250535392,
114.376547448128,114.406671945289),.UNSPECIFIED.);
#1017=B_SPLINE_CURVE_WITH_KNOTS('',3,(#104369,#104370,#104371,#104372,#104373,
#104374,#104375,#104376,#104377,#104378),.UNSPECIFIED.,.F.,.F.,(4,1,1,1,
1,1,1,4),(114.406674973168,114.866191745616,115.865028195577,116.863864645539,
117.862701095501,118.861537545463,119.860373995425,120.339865682355),
 .UNSPECIFIED.);
#1018=B_SPLINE_CURVE_WITH_KNOTS('',3,(#104379,#104380,#104381,#104382,#104383,
#104384,#104385,#104386,#104387,#104388,#104389,#104390,#104391,#104392,
#104393,#104394,#104395,#104396,#104397,#104398,#104399,#104400,#104401,
#104402,#104403,#104404,#104405,#104406,#104407,#104408,#104409,#104410,
#104411,#104412,#104413,#104414,#104415,#104416,#104417,#104418,#104419,
#104420,#104421,#104422,#104423,#104424,#104425,#104426,#104427,#104428,
#104429,#104430,#104431,#104432,#104433,#104434,#104435,#104436,#104437,
#104438,#104439,#104440,#104441,#104442,#104443,#104444,#104445,#104446,
#104447,#104448,#104449,#104450,#104451,#104452,#104453,#104454,#104455,
#104456,#104457,#104458,#104459,#104460,#104461,#104462,#104463,#104464,
#104465,#104466,#104467,#104468,#104469,#104470,#104471,#104472,#104473,
#104474,#104475,#104476,#104477,#104478,#104479,#104480,#104481,#104482,
#104483,#104484,#104485,#104486,#104487,#104488,#104489,#104490,#104491,
#104492,#104493,#104494,#104495,#104496,#104497,#104498,#104499,#104500,
#104501,#104502,#104503,#104504,#104505,#104506,#104507,#104508,#104509,
#104510,#104511,#104512,#104513,#104514,#104515,#104516,#104517,#104518,
#104519,#104520,#104521,#104522,#104523,#104524,#104525,#104526,#104527,
#104528,#104529,#104530,#104531,#104532,#104533,#104534,#104535,#104536,
#104537,#104538,#104539,#104540,#104541,#104542,#104543,#104544,#104545,
#104546,#104547,#104548,#104549,#104550,#104551,#104552,#104553,#104554,
#104555,#104556,#104557,#104558,#104559,#104560,#104561,#104562,#104563,
#104564,#104565,#104566,#104567,#104568,#104569,#104570,#104571,#104572,
#104573,#104574,#104575,#104576,#104577,#104578,#104579,#104580,#104581,
#104582,#104583,#104584,#104585,#104586,#104587,#104588,#104589,#104590,
#104591,#104592,#104593,#104594,#104595,#104596,#104597,#104598,#104599,
#104600,#104601,#104602,#104603,#104604,#104605,#104606,#104607,#104608,
#104609,#104610,#104611,#104612,#104613,#104614,#104615,#104616,#104617,
#104618,#104619,#104620,#104621,#104622,#104623,#104624,#104625,#104626,
#104627,#104628,#104629,#104630,#104631,#104632,#104633,#104634,#104635,
#104636,#104637,#104638,#104639,#104640,#104641,#104642,#104643,#104644),
 .UNSPECIFIED.,.F.,.F.,(4,2,2,2,2,2,2,2,2,2,2,2,2,2,2,2,2,2,2,2,2,2,2,2,
2,2,2,2,2,2,2,2,2,2,2,2,2,2,2,2,2,2,2,2,2,2,2,2,2,2,2,2,2,2,2,2,2,2,2,2,
2,2,2,2,2,2,2,2,2,2,2,2,2,2,2,2,2,2,2,2,2,2,2,2,2,2,2,2,2,2,2,2,2,2,2,2,
2,2,2,2,2,2,2,2,2,2,2,2,2,2,2,2,2,2,2,2,2,2,2,2,2,2,2,2,2,2,2,2,2,2,2,2,
4),(-2.59392646598523,-2.58066502555958,-2.56300901345937,-2.5522099013361,
-2.54890542051214,-2.54681924632914,-2.54488227583739,-2.54236837323655,
-2.5381689719236,-2.50879236248568,-2.46759283265409,-2.45213649756508,
-2.44671689522576,-2.44411614220636,-2.44200814993706,-2.44079506757119,
-2.44079195659206,-2.44078882665356,-2.44078567760298,-2.44078250933715,
-2.44077932176747,-2.44077611469552,-2.44077288804981,-2.44076964168511,
-2.44076637548386,-2.44076308927576,-2.4407597829211,-2.44075645626122,
-2.44075312209097,-2.44074977343357,-2.44074640360696,-2.44074301250016,
-2.44073958889878,-2.43971148371076,-2.43833172623461,-2.43546361523069,
-2.39998403574502,-2.36704576945719,-2.34422233712747,-2.3385327789589,
-2.33595465332513,-2.33401488516542,-2.33218976179598,-2.32965454379678,
-2.32305751480103,-2.2667982738266,-2.24302124160745,-2.23227440562075,
-2.23003480513183,-2.22878538166568,-2.22771312142934,-2.22635539967584,
-2.22420476539108,-2.21309029939523,-2.1618232717555,-2.13321419439624,
-2.12679182067121,-2.12408473194876,-2.12212305523122,-2.12032966709056,
-2.11746177027316,-2.11056132915635,-2.05766974361515,-2.03162195559925,
-2.02027804318085,-2.01800314045304,-2.0167460504074,-2.01567454060791,
-2.01432710904692,-2.01170759989892,-1.99570618493379,-1.99020645925097,
-1.97577391529199,-1.94287710523563,-1.92630900304767,-1.91599546283168,
-1.91274595649969,-1.91067212434943,-1.90873096721912,-1.90618916869418,
-1.90189311034052,-1.86675840593335,-1.81779579351645,-1.80808008488306,
-1.80590731934123,-1.80467250585235,-1.80359837273467,-1.8022194686122,
-1.79935615455937,-1.76334935722691,-1.73058682285606,-1.70804069402824,
-1.7023882896687,-1.69981682302094,-1.69787792662867,-1.69605058389674,
-1.69350740843637,-1.68686090440254,-1.63107000103531,-1.59817517576441,
-1.59462811060725,-1.59312359316423,-1.59203199788474,-1.59100445649406,
-1.58925398277654,-1.58447447185232,-1.54730070324189,-1.49702116171413,
-1.49061825743434,-1.48791429555067,-1.48595303431212,-1.48415875065031,
-1.48128664121933,-1.47436166830793,-1.421787532311,-1.39551110069199,-1.38410882121919,
-1.38183041999204,-1.38057249260765,-1.3795009329836,-1.37815428305887,
-1.37553877115204,-1.35961660813774,-1.35511411290143,-1.33454900263241,
-1.28619023022274,-1.27904054767369,-1.27613103133974,-1.27432986351377,
-1.27237413797995,-1.26970141794458,-1.26348138904713,-1.26001305103131),
 .UNSPECIFIED.);
#1019=B_SPLINE_CURVE_WITH_KNOTS('',3,(#104650,#104651,#104652,#104653,#104654,
#104655,#104656,#104657,#104658,#104659,#104660,#104661,#104662,#104663,
#104664,#104665,#104666,#104667,#104668,#104669),.UNSPECIFIED.,.F.,.F.,
(4,2,2,2,2,2,2,2,2,4),(-0.0747504621130409,-0.0610229394801576,-0.0562870045128616,
-0.054543581138797,-0.0535177052337252,-0.0524257925231619,-0.0509174394464196,
-0.0492296206923426,-0.0462824100167693,-0.000629119177008705),
 .UNSPECIFIED.);
#1020=B_SPLINE_CURVE_WITH_KNOTS('',3,(#104670,#104671,#104672,#104673,#104674,
#104675,#104676,#104677,#104678,#104679,#104680,#104681,#104682,#104683,
#104684,#104685,#104686,#104687,#104688,#104689,#104690,#104691,#104692,
#104693,#104694,#104695,#104696,#104697,#104698,#104699,#104700,#104701,
#104702,#104703,#104704,#104705,#104706,#104707,#104708,#104709,#104710,
#104711,#104712,#104713,#104714,#104715,#104716,#104717,#104718,#104719,
#104720,#104721,#104722,#104723,#104724,#104725,#104726,#104727,#104728,
#104729,#104730,#104731,#104732,#104733,#104734,#104735,#104736,#104737,
#104738,#104739,#104740,#104741,#104742,#104743,#104744,#104745,#104746,
#104747,#104748,#104749,#104750,#104751,#104752,#104753,#104754,#104755,
#104756,#104757,#104758,#104759,#104760,#104761,#104762,#104763,#104764,
#104765,#104766,#104767,#104768,#104769,#104770,#104771,#104772,#104773,
#104774,#104775,#104776,#104777,#104778,#104779,#104780,#104781,#104782,
#104783,#104784,#104785,#104786,#104787,#104788,#104789,#104790,#104791,
#104792,#104793,#104794,#104795,#104796,#104797,#104798,#104799,#104800,
#104801,#104802,#104803,#104804,#104805,#104806,#104807,#104808,#104809,
#104810,#104811,#104812,#104813,#104814,#104815,#104816,#104817,#104818,
#104819,#104820,#104821,#104822,#104823,#104824,#104825,#104826,#104827,
#104828,#104829,#104830,#104831,#104832,#104833,#104834,#104835,#104836,
#104837,#104838,#104839,#104840,#104841,#104842,#104843,#104844,#104845,
#104846,#104847,#104848,#104849,#104850),.UNSPECIFIED.,.F.,.F.,(4,3,3,3,
3,3,3,3,3,3,3,3,3,3,3,3,3,3,3,3,3,3,3,3,3,3,3,3,3,3,3,3,3,3,3,3,3,3,3,3,
3,3,3,3,3,3,3,3,3,3,3,3,3,3,3,3,3,3,3,3,4),(108.12348663811,108.225421296431,
108.327291076165,108.429131491865,108.530978014042,108.632930880403,108.734945943836,
108.837130903885,108.873173045844,108.976567782892,109.079809065007,109.1829290304,
109.285983598609,109.389006806967,109.492032649639,109.595165416417,109.698354507827,
109.801726501209,109.872009495806,109.975404232854,110.078645514969,110.181765480362,
110.28482004857,110.387843256928,110.490869099601,110.594001866379,110.697190957789,
110.800562951171,110.870845945768,110.974240682816,111.077481964931,111.180601930323,
111.283656498532,111.38667970689,111.489705549562,111.59283831634,111.69602740775,
111.799399401132,111.86968239573,111.973077132778,112.076318414893,112.179438380285,
112.282492948494,112.385516156852,112.488541999524,112.591674766303,112.694863857712,
112.798235851094,112.868518845692,112.97191358274,113.075154864855,113.178274830248,
113.281329398457,113.384352606815,113.487378449487,113.590511216265,113.693700307675,
113.797072301057,113.867355295654,113.974272639368,114.057240443604),
 .UNSPECIFIED.);
#1021=B_SPLINE_CURVE_WITH_KNOTS('',3,(#104852,#104853,#104854,#104855,#104856,
#104857,#104858,#104859,#104860,#104861,#104862,#104863,#104864,#104865,
#104866,#104867,#104868,#104869,#104870,#104871,#104872,#104873,#104874,
#104875,#104876,#104877,#104878,#104879,#104880,#104881,#104882,#104883,
#104884,#104885,#104886,#104887,#104888,#104889,#104890,#104891,#104892,
#104893,#104894,#104895,#104896,#104897,#104898,#104899,#104900,#104901,
#104902,#104903,#104904,#104905,#104906,#104907,#104908,#104909,#104910,
#104911,#104912,#104913,#104914,#104915,#104916,#104917,#104918,#104919,
#104920,#104921,#104922,#104923,#104924,#104925,#104926,#104927,#104928,
#104929,#104930,#104931,#104932,#104933,#104934,#104935,#104936,#104937,
#104938,#104939,#104940,#104941,#104942,#104943,#104944,#104945,#104946,
#104947,#104948,#104949,#104950,#104951,#104952,#104953,#104954,#104955,
#104956,#104957,#104958,#104959,#104960,#104961,#104962,#104963,#104964,
#104965,#104966,#104967,#104968,#104969,#104970,#104971,#104972,#104973,
#104974,#104975,#104976,#104977,#104978,#104979,#104980,#104981,#104982,
#104983,#104984,#104985,#104986,#104987,#104988,#104989,#104990,#104991,
#104992,#104993,#104994,#104995,#104996,#104997,#104998,#104999,#105000,
#105001,#105002,#105003,#105004,#105005,#105006,#105007,#105008,#105009,
#105010,#105011,#105012,#105013,#105014,#105015,#105016,#105017,#105018,
#105019,#105020,#105021,#105022,#105023,#105024,#105025,#105026,#105027,
#105028,#105029,#105030,#105031,#105032,#105033,#105034,#105035,#105036,
#105037,#105038,#105039,#105040,#105041,#105042,#105043,#105044,#105045,
#105046,#105047,#105048,#105049,#105050,#105051,#105052,#105053,#105054,
#105055,#105056,#105057,#105058,#105059,#105060,#105061,#105062,#105063,
#105064,#105065,#105066,#105067),.UNSPECIFIED.,.F.,.F.,(4,2,2,2,2,2,2,2,
2,2,2,2,2,2,2,2,2,2,2,2,2,2,2,2,2,2,2,2,2,2,2,2,2,2,2,2,2,2,2,2,2,2,2,2,
2,2,2,2,2,2,2,2,2,2,2,2,2,2,2,2,2,2,2,2,2,2,2,2,2,2,2,2,2,2,2,2,2,2,2,2,
2,2,2,2,2,2,2,2,2,2,2,2,2,2,2,2,2,2,2,2,2,2,2,2,2,2,2,4),(-1.26001305103131,
-1.236546528138,-1.19601723368554,-1.17302338979252,-1.17016774612471,-1.1687903357867,
-1.16771632918863,-1.1664804986667,-1.16430315072426,-1.15452122247037,
-1.10558802777883,-1.0704579529701,-1.06616178556445,-1.06361998936534,
-1.06167886157342,-1.05960508658686,-1.05635572252675,-1.0460429935662,
-1.02947884433227,-0.996613617850608,-0.982869511029417,-0.976019436372951,
-0.97570881818813,-0.970189105870943,-0.960125838630565,-0.958043063190949,
-0.956706143309467,-0.955635277538568,-0.954369928227707,-0.952056799877416,
-0.940020236017337,-0.888050633906243,-0.858275267555108,-0.854081820408176,
-0.851570075538851,-0.849633932071001,-0.847547823011974,-0.844241681169512,
-0.8334212373689,-0.815716956570843,-0.765142043162348,-0.748688316661077,
-0.746050663149659,-0.744699388111575,-0.74362769297481,-0.742373709538034,
-0.740112823948655,-0.729008814736019,-0.703888241194228,-0.649614579223858,
-0.642824912843948,-0.639975427925457,-0.638185470213055,-0.636221016593174,
-0.633498051885379,-0.626980395416872,-0.597568275097048,-0.547613731328803,
-0.536213183438616,-0.534045464982643,-0.532682628984102,-0.531610088504744,
-0.530364645439957,-0.528142810196855,-0.517678996270604,-0.494920901946999,
-0.437029625182237,-0.430618952160738,-0.428114251199299,-0.426297280064509,
-0.424353285136179,-0.421747270802334,-0.41590291347179,-0.391914313035495,
-0.342043705642979,-0.32466688567579,-0.321994678619817,-0.320636069225288,
-0.31956391413444,-0.318315545180878,-0.316080138974597,-0.305397394370176,
-0.28184949767725,-0.225205284497385,-0.218651621412212,-0.215899096865799,
-0.21395697617716,-0.212008337317596,-0.21003265608343,-0.204809495390636,
-0.197989211077535,-0.181524624333188,-0.14874670231778,-0.112915186594562,
-0.110056468619816,-0.108678728269664,-0.107605005720207,-0.106370113057628,
-0.104195878191195,-0.094452065454749,-0.0455058292351705,-0.0267279147051765,
-0.018764008653592,-0.00802108915905755,-0.00466632909900502,-0.00258130056107843,
-0.00128118359696819,-0.000628940766197544),.UNSPECIFIED.);
#1022=B_SPLINE_CURVE_WITH_KNOTS('',3,(#105068,#105069,#105070,#105071,#105072,
#105073,#105074,#105075,#105076,#105077,#105078,#105079,#105080),
 .UNSPECIFIED.,.F.,.F.,(4,3,3,3,4),(-104.372003947921,-104.263735348745,
-104.155311094227,-104.046631225742,-104.02252548323),.UNSPECIFIED.);
#1023=B_SPLINE_CURVE_WITH_KNOTS('',3,(#105085,#105086,#105087,#105088,#105089,
#105090,#105091,#105092,#105093,#105094,#105095,#105096,#105097,#105098,
#105099,#105100,#105101,#105102,#105103,#105104,#105105,#105106,#105107,
#105108,#105109,#105110,#105111,#105112,#105113,#105114,#105115,#105116,
#105117,#105118,#105119,#105120,#105121,#105122,#105123,#105124,#105125,
#105126,#105127,#105128,#105129,#105130,#105131,#105132,#105133,#105134,
#105135,#105136,#105137,#105138,#105139,#105140,#105141,#105142,#105143,
#105144,#105145,#105146,#105147,#105148,#105149,#105150,#105151,#105152,
#105153,#105154,#105155,#105156,#105157,#105158,#105159,#105160,#105161,
#105162,#105163,#105164,#105165,#105166,#105167,#105168,#105169,#105170,
#105171,#105172,#105173,#105174,#105175,#105176,#105177,#105178,#105179,
#105180,#105181,#105182,#105183,#105184,#105185,#105186,#105187,#105188,
#105189,#105190,#105191,#105192,#105193,#105194,#105195,#105196,#105197,
#105198,#105199,#105200,#105201,#105202,#105203,#105204,#105205,#105206,
#105207,#105208,#105209,#105210,#105211,#105212,#105213,#105214,#105215,
#105216,#105217,#105218,#105219,#105220,#105221,#105222,#105223,#105224,
#105225,#105226,#105227,#105228,#105229,#105230,#105231,#105232,#105233,
#105234,#105235,#105236,#105237,#105238,#105239,#105240,#105241,#105242,
#105243,#105244,#105245,#105246,#105247,#105248,#105249,#105250,#105251,
#105252,#105253,#105254,#105255,#105256,#105257,#105258,#105259,#105260,
#105261,#105262,#105263,#105264,#105265,#105266,#105267,#105268,#105269,
#105270,#105271,#105272,#105273,#105274,#105275,#105276,#105277,#105278,
#105279,#105280,#105281,#105282,#105283,#105284,#105285,#105286,#105287,
#105288,#105289,#105290,#105291,#105292,#105293,#105294,#105295,#105296,
#105297,#105298,#105299,#105300,#105301,#105302,#105303,#105304),
 .UNSPECIFIED.,.F.,.F.,(4,2,2,2,2,2,2,2,2,2,2,2,2,2,2,2,2,2,2,2,2,2,2,2,
2,2,2,2,2,2,2,2,2,2,2,2,2,2,2,2,2,2,2,2,2,2,2,2,2,2,2,2,2,2,2,2,2,2,2,2,
2,2,2,2,2,2,2,2,2,2,2,2,2,2,2,2,2,2,2,2,2,2,2,2,2,2,2,2,2,2,2,2,2,2,2,2,
2,2,2,2,2,2,2,2,2,2,2,2,2,4),(-1.40835486065175,-1.37307255299345,-1.33396207864897,
-1.33297748426174,-1.32826979514078,-1.32653032040276,-1.32550499424266,
-1.32441216338815,-1.32290008987306,-1.31930843874777,-1.28016662750195,
-1.231343669678,-1.22421240551894,-1.22130614945658,-1.21950571100321,-1.21754975931901,
-1.21487489659208,-1.20864151528037,-1.18159595652532,-1.14086971316094,
-1.11820870358814,-1.11535575851077,-1.11397896091013,-1.11290510797361,
-1.11166908812003,-1.1094905298683,-1.09968861468525,-1.05077804374086,
-1.01565733058686,-1.0113616749969,-1.00882015837761,-1.00687923071736,
-1.00480565656637,-1.00155658010668,-0.991244535586352,-0.974681268546033,
-0.941818709324578,-0.928012119514121,-0.921312903073065,-0.90586503211797,
-0.903497117398427,-0.902089535649802,-0.901009379508387,-0.899805930223189,
-0.89777412752424,-0.889883895692131,-0.875166680607255,-0.846103611921341,
-0.803698157867828,-0.799404688363424,-0.796863862447183,-0.79492311507512,
-0.792849396808795,-0.78959939123828,-0.779278464535908,-0.762695283424875,
-0.72981705058985,-0.714520484150677,-0.709793773457523,-0.693941561266164,
-0.691328748893703,-0.689982891873249,-0.688911647907598,-0.687653730774862,
-0.685374419137727,-0.673948877877966,-0.647572472915313,-0.595122291163116,
-0.58818879175417,-0.585315747503484,-0.583521640547718,-0.581561188059488,
-0.578859459016999,-0.572467089056242,-0.526046822988734,-0.484947942418818,
-0.480263095535808,-0.478527315143957,-0.477502864635007,-0.476409860217495,
-0.474895738211797,-0.471290870983224,-0.432949505047567,-0.383317401821813,
-0.376221669184502,-0.373321738335967,-0.371522744055547,-0.36956640256799,
-0.366887471566432,-0.360806609691591,-0.352445821237174,-0.301551441055394,
-0.270313241009477,-0.267401273969782,-0.266013097090093,-0.264938281360049,
-0.263710016435639,-0.26156604738355,-0.252414963132737,-0.203666416644472,
-0.167704289861289,-0.162982355971044,-0.160559557536596,-0.158640676069439,
-0.156487802200587,-0.154258046820985,-0.146612093912555,-0.121083043579651,
-0.100337615416932,-0.0747504621130409),.UNSPECIFIED.);
#1024=B_SPLINE_CURVE_WITH_KNOTS('',3,(#105306,#105307,#105308,#105309,#105310,
#105311,#105312,#105313,#105314,#105315,#105316,#105317,#105318,#105319,
#105320,#105321,#105322,#105323,#105324,#105325,#105326,#105327,#105328,
#105329,#105330,#105331,#105332,#105333,#105334,#105335,#105336,#105337,
#105338,#105339,#105340,#105341,#105342,#105343,#105344,#105345,#105346,
#105347,#105348,#105349,#105350,#105351,#105352,#105353,#105354,#105355,
#105356,#105357,#105358,#105359,#105360,#105361,#105362,#105363,#105364,
#105365,#105366,#105367,#105368,#105369,#105370,#105371,#105372,#105373,
#105374,#105375,#105376,#105377,#105378,#105379,#105380,#105381,#105382,
#105383,#105384,#105385,#105386,#105387,#105388,#105389,#105390,#105391,
#105392,#105393,#105394,#105395,#105396,#105397,#105398,#105399,#105400,
#105401,#105402,#105403,#105404,#105405,#105406,#105407,#105408,#105409,
#105410,#105411,#105412,#105413,#105414,#105415,#105416,#105417,#105418,
#105419,#105420,#105421,#105422,#105423,#105424,#105425,#105426,#105427,
#105428,#105429,#105430,#105431,#105432,#105433,#105434,#105435,#105436,
#105437,#105438,#105439,#105440,#105441,#105442,#105443,#105444,#105445,
#105446,#105447,#105448,#105449,#105450,#105451,#105452,#105453,#105454,
#105455,#105456,#105457,#105458,#105459,#105460,#105461,#105462,#105463,
#105464,#105465,#105466,#105467,#105468,#105469,#105470,#105471,#105472,
#105473,#105474,#105475,#105476,#105477,#105478,#105479,#105480,#105481,
#105482,#105483,#105484,#105485,#105486),.UNSPECIFIED.,.F.,.F.,(4,3,3,3,
3,3,3,3,3,3,3,3,3,3,3,3,3,3,3,3,3,3,3,3,3,3,3,3,3,3,3,3,3,3,3,3,3,3,3,3,
3,3,3,3,3,3,3,3,3,3,3,3,3,3,3,3,3,3,3,3,4),(-104.02252548323,-103.91351434008,
-103.878990796035,-103.775596058987,-103.672354776872,-103.569234811479,
-103.46618024327,-103.363157034913,-103.26013119224,-103.156998425462,-103.053809334052,
-102.95043734067,-102.880154346073,-102.776759609025,-102.67351832691,-102.570398361518,
-102.467343793309,-102.364320584951,-102.261294742278,-102.1581619755,-102.05497288409,
-101.951600890709,-101.881317896111,-101.777923159063,-101.674681876948,
-101.571561911556,-101.468507343347,-101.365484134989,-101.262458292316,
-101.159325525538,-101.056136434129,-100.952764440747,-100.882481446149,
-100.779086709101,-100.675845426986,-100.572725461594,-100.469670893385,
-100.366647685027,-100.263621842355,-100.160489075577,-100.057299984167,
-99.9539279907855,-99.8836449961874,-99.7802502591395,-99.6770089770246,
-99.5738890116323,-99.4708344434234,-99.3678112350657,-99.2647853923932,
-99.1616526256152,-99.0584635342055,-98.9550915408238,-98.8848085462255,
-98.7829332776307,-98.681193284401,-98.5795525376358,-98.4779751499171,
-98.3763829554481,-98.2747883682232,-98.173080529173,-98.088818832803),
 .UNSPECIFIED.);
#1025=B_SPLINE_CURVE_WITH_KNOTS('',3,(#105487,#105488,#105489,#105490,#105491),
 .UNSPECIFIED.,.F.,.F.,(4,1,4),(-98.0888186411165,-97.8859720962637,-97.7379483482805),
 .UNSPECIFIED.);
#1026=B_SPLINE_CURVE_WITH_KNOTS('',3,(#105497,#105498,#105499,#105500,#105501,
#105502,#105503,#105504,#105505,#105506,#105507,#105508,#105509,#105510,
#105511,#105512,#105513,#105514,#105515,#105516,#105517,#105518),
 .UNSPECIFIED.,.F.,.F.,(4,2,2,2,2,2,2,2,2,2,4),(-0.0750516936837853,-0.0634020284095776,
-0.0604358780118531,-0.0436144741885916,-0.039999552682271,-0.0376361154365763,
-0.0357225173379457,-0.0339209980332159,-0.0317709111716201,-0.028634281768215,
-0.00062847532083142),.UNSPECIFIED.);
#1027=B_SPLINE_CURVE_WITH_KNOTS('',3,(#105519,#105520,#105521,#105522,#105523,
#105524,#105525,#105526,#105527,#105528,#105529,#105530,#105531,#105532,
#105533,#105534,#105535,#105536,#105537,#105538,#105539,#105540,#105541,
#105542,#105543,#105544,#105545,#105546,#105547,#105548,#105549,#105550,
#105551,#105552,#105553,#105554,#105555,#105556,#105557,#105558,#105559,
#105560,#105561,#105562,#105563,#105564,#105565,#105566,#105567,#105568,
#105569,#105570,#105571,#105572,#105573,#105574,#105575,#105576,#105577,
#105578,#105579,#105580,#105581,#105582,#105583,#105584,#105585,#105586,
#105587,#105588,#105589,#105590,#105591,#105592,#105593,#105594,#105595,
#105596,#105597,#105598,#105599,#105600,#105601,#105602,#105603,#105604,
#105605,#105606,#105607,#105608,#105609,#105610,#105611,#105612,#105613,
#105614,#105615,#105616,#105617,#105618,#105619,#105620,#105621,#105622,
#105623,#105624,#105625,#105626,#105627,#105628,#105629,#105630,#105631,
#105632,#105633,#105634,#105635,#105636,#105637,#105638,#105639,#105640,
#105641,#105642,#105643,#105644,#105645,#105646,#105647,#105648,#105649,
#105650,#105651,#105652,#105653,#105654,#105655,#105656,#105657,#105658,
#105659,#105660,#105661,#105662,#105663,#105664,#105665,#105666,#105667,
#105668,#105669,#105670,#105671,#105672,#105673,#105674,#105675,#105676,
#105677,#105678,#105679,#105680,#105681,#105682,#105683,#105684,#105685,
#105686,#105687,#105688,#105689,#105690,#105691,#105692,#105693,#105694,
#105695,#105696,#105697,#105698,#105699,#105700,#105701,#105702,#105703,
#105704,#105705,#105706,#105707,#105708,#105709,#105710,#105711,#105712,
#105713,#105714,#105715,#105716,#105717,#105718,#105719,#105720,#105721,
#105722,#105723,#105724,#105725,#105726,#105727,#105728,#105729,#105730,
#105731,#105732,#105733,#105734,#105735,#105736),.UNSPECIFIED.,.F.,.F.,
(4,2,2,2,2,2,2,2,2,2,2,2,2,2,2,2,2,2,2,2,2,2,2,2,2,2,2,2,2,2,2,2,2,2,2,
2,2,2,2,2,2,2,2,2,2,2,2,2,2,2,2,2,2,2,2,2,2,2,2,2,2,2,2,2,2,2,2,2,2,2,2,
2,2,2,2,2,2,2,2,2,2,2,2,2,2,2,2,2,2,2,2,2,2,2,2,2,2,2,2,2,2,2,2,2,2,2,2,
2,4),(-2.66765111215731,-2.62407445969734,-2.60409385631716,-2.60009969993428,
-2.59852161183882,-2.59741658343656,-2.59640713873932,-2.59474984029436,
-2.59056385451666,-2.54053209371147,-2.51638356999891,-2.50455767987239,
-2.49657807409339,-2.49363506596365,-2.49184383953861,-2.48990306162119,
-2.48736308345081,-2.48307306618434,-2.44794206582757,-2.39901908258442,
-2.38926017550042,-2.38708452483878,-2.38584911720301,-2.38477513702998,
-2.38339730507794,-2.38053923481449,-2.35767518797266,-2.31214656554528,
-2.29549076408549,-2.28513772404252,-2.28188377473653,-2.27980902410011,
-2.27786835206758,-2.27532912684878,-2.27104175607711,-2.23592408342776,
-2.18705567479819,-2.17723123233823,-2.17505109491602,-2.17381469258006,
-2.17274084029038,-2.1713644687973,-2.16851388094193,-2.13210984678009,
-2.07830554016108,-2.07184821374121,-2.06913522816466,-2.06717247666518,
-2.06538030292746,-2.06251912043925,-2.05565952917868,-2.00224248325543,
-1.97655925428298,-1.96530844930874,-1.96303890217495,-1.96178297358227,
-1.96071136080605,-1.9593624071158,-1.95673583757679,-1.94056643275142,
-1.93131628638674,-1.89233774568212,-1.86585604079635,-1.85969287225457,
-1.85703013956307,-1.85507628727629,-1.85327303306179,-1.8503516278065,
-1.84313034462125,-1.79864231564355,-1.78473362850401,-1.76327602592312,
-1.75318370090961,-1.75098566897263,-1.74974535124647,-1.74867204967684,
-1.74730152130014,-1.74510870590138,-1.73333923482992,-1.72962683247937,
-1.72236557804097,-1.67901009360733,-1.66042268654731,-1.64921987837732,
-1.64587221629192,-1.6437768023276,-1.64184353018162,-1.63935164944882,
-1.63522643606853,-1.60809056910824,-1.56616637828247,-1.54954737000885,
-1.5409847878197,-1.53889723711027,-1.53768129815543,-1.53660390598313,
-1.53521798115663,-1.53292427491676,-1.51915033083512,-1.50784478798864,
-1.46844818216272,-1.44187538096531,-1.43570086894304,-1.43303616072426,
-1.43108195985373,-1.42927915700106,-1.42636021023468,-1.419153546198,-1.40835486065175),
 .UNSPECIFIED.);
#1028=B_SPLINE_CURVE_WITH_KNOTS('',3,(#105738,#105739,#105740,#105741,#105742,
#105743,#105744,#105745,#105746,#105747),.UNSPECIFIED.,.F.,.F.,(4,1,1,1,
1,1,1,4),(-97.7379483482805,-96.8871356463018,-95.8882991963399,-94.889462746378,
-93.8906262964161,-92.8917898464543,-91.8929533964924,-91.8056333339369),
 .UNSPECIFIED.);
#1029=B_SPLINE_CURVE_WITH_KNOTS('',3,(#105748,#105749,#105750,#105751,#105752,
#105753,#105754,#105755),.UNSPECIFIED.,.F.,.F.,(4,2,2,4),(-2.66796196902112,
-2.61567753669294,-2.59732738807453,-2.59351319560632),.UNSPECIFIED.);
#1030=B_SPLINE_CURVE_WITH_KNOTS('',3,(#105760,#105761,#105762,#105763,#105764,
#105765,#105766,#105767,#105768,#105769,#105770,#105771,#105772,#105773,
#105774,#105775,#105776,#105777,#105778,#105779,#105780,#105781,#105782,
#105783,#105784,#105785,#105786,#105787,#105788,#105789,#105790,#105791,
#105792,#105793,#105794,#105795,#105796,#105797,#105798,#105799,#105800,
#105801,#105802,#105803,#105804,#105805,#105806,#105807,#105808,#105809,
#105810,#105811,#105812,#105813,#105814,#105815,#105816,#105817,#105818,
#105819,#105820,#105821,#105822,#105823,#105824,#105825,#105826,#105827,
#105828,#105829,#105830,#105831,#105832,#105833,#105834,#105835,#105836,
#105837,#105838,#105839,#105840,#105841,#105842,#105843,#105844,#105845,
#105846,#105847,#105848,#105849,#105850,#105851,#105852,#105853,#105854,
#105855,#105856,#105857,#105858,#105859,#105860,#105861,#105862,#105863,
#105864,#105865,#105866,#105867,#105868,#105869,#105870,#105871,#105872,
#105873,#105874,#105875,#105876,#105877,#105878,#105879,#105880,#105881,
#105882,#105883,#105884,#105885,#105886,#105887,#105888,#105889,#105890,
#105891,#105892,#105893,#105894,#105895,#105896,#105897,#105898,#105899,
#105900,#105901,#105902,#105903,#105904,#105905,#105906,#105907,#105908,
#105909,#105910,#105911,#105912,#105913,#105914,#105915,#105916,#105917,
#105918,#105919,#105920,#105921,#105922,#105923,#105924,#105925,#105926,
#105927,#105928,#105929,#105930,#105931,#105932,#105933,#105934,#105935,
#105936,#105937,#105938,#105939,#105940,#105941,#105942,#105943,#105944,
#105945,#105946,#105947,#105948,#105949,#105950,#105951,#105952,#105953,
#105954,#105955,#105956,#105957,#105958,#105959,#105960,#105961,#105962,
#105963,#105964,#105965,#105966,#105967,#105968,#105969,#105970,#105971,
#105972,#105973,#105974,#105975),.UNSPECIFIED.,.F.,.F.,(4,2,2,2,2,2,2,2,
2,2,2,2,2,2,2,2,2,2,2,2,2,2,2,2,2,2,2,2,2,2,2,2,2,2,2,2,2,2,2,2,2,2,2,2,
2,2,2,2,2,2,2,2,2,2,2,2,2,2,2,2,2,2,2,2,2,2,2,2,2,2,2,2,2,2,2,2,2,2,2,2,
2,2,2,2,2,2,2,2,2,2,2,2,2,2,2,2,2,2,2,2,2,2,2,2,2,2,2,4),(-1.40856975518855,
-1.37753587866969,-1.33437708927627,-1.31573942604955,-1.31200670593019,
-1.30960679601331,-1.30769002652343,-1.30552247328272,-1.30184787503229,
-1.28708495689693,-1.25915990071243,-1.20936296122167,-1.20516000691329,
-1.20350003174228,-1.20249023890662,-1.20138599617114,-1.19981100945422,
-1.19583510293771,-1.17602243210622,-1.14710962007291,-1.10479066552403,
-1.10049554998527,-1.09795430887023,-1.09601356625899,-1.09394016522393,
-1.09069130869549,-1.08037952948746,-1.06381627701968,-1.03095548478581,
-1.01703050932108,-1.01060171826353,-0.995018249780802,-0.992416681650823,
-0.991073289507136,-0.990002246656862,-0.988742517785766,-0.986454683199814,
-0.974876354420389,-0.94788591706954,-0.896303999186155,-0.889313147946355,
-0.886430715237282,-0.884634956267085,-0.882676062091122,-0.879982610669475,
-0.873638510385787,-0.845679555567062,-0.799181399229366,-0.78306901187068,
-0.780442219249276,-0.779093411635139,-0.778022051023146,-0.776766581434501,
-0.774498267217136,-0.763262292897871,-0.737629700058277,-0.684119355716797,
-0.677267312166131,-0.674407802274688,-0.672616250976325,-0.670653844248833,
-0.667940707904399,-0.661480017710091,-0.607515332483881,-0.571349700551674,
-0.568494221403407,-0.56711711175029,-0.566043443635467,-0.564808120067418,
-0.562631946360587,-0.552859947082846,-0.503937170129568,-0.468830136471749,
-0.464527892189037,-0.461984761505626,-0.460043915174238,-0.457971700664554,
-0.454727409177611,-0.444452873120169,-0.427971021338313,-0.371279173650671,
-0.358728321248603,-0.356496629706004,-0.355114537874551,-0.354040395715363,
-0.352808363303963,-0.350647107763793,-0.341090377556351,-0.291984792241839,
-0.256812528772424,-0.252513924435505,-0.249971864513634,-0.248031213376732,
-0.246240564164274,-0.243303252798097,-0.235329252280526,-0.223526490989541,
-0.190999838568903,-0.150078388071853,-0.14538763422155,-0.143651112007467,
-0.142626619777758,-0.141533907642915,-0.140020740693023,-0.136420690088568,
-0.098526352753562,-0.0757357784074703,-0.0750516936837853),
 .UNSPECIFIED.);
#1031=B_SPLINE_CURVE_WITH_KNOTS('',3,(#105976,#105977,#105978,#105979,#105980,
#105981,#105982,#105983,#105984,#105985,#105986,#105987,#105988,#105989,
#105990,#105991,#105992,#105993,#105994,#105995,#105996,#105997,#105998,
#105999,#106000,#106001,#106002,#106003,#106004,#106005,#106006,#106007,
#106008,#106009,#106010,#106011,#106012,#106013,#106014,#106015,#106016,
#106017,#106018,#106019,#106020,#106021,#106022,#106023,#106024,#106025,
#106026,#106027,#106028,#106029,#106030,#106031,#106032,#106033,#106034,
#106035,#106036,#106037,#106038,#106039,#106040,#106041,#106042,#106043,
#106044,#106045,#106046,#106047,#106048,#106049,#106050,#106051,#106052,
#106053,#106054,#106055,#106056,#106057,#106058,#106059,#106060,#106061,
#106062,#106063,#106064,#106065,#106066,#106067,#106068,#106069,#106070,
#106071,#106072,#106073,#106074,#106075,#106076,#106077,#106078,#106079,
#106080,#106081,#106082,#106083,#106084,#106085,#106086,#106087,#106088,
#106089,#106090,#106091,#106092,#106093,#106094,#106095,#106096,#106097,
#106098,#106099,#106100,#106101,#106102,#106103,#106104,#106105,#106106,
#106107,#106108,#106109,#106110,#106111,#106112,#106113,#106114,#106115,
#106116,#106117,#106118,#106119,#106120,#106121,#106122,#106123,#106124,
#106125,#106126,#106127,#106128,#106129,#106130,#106131,#106132,#106133,
#106134,#106135,#106136,#106137,#106138,#106139,#106140,#106141,#106142,
#106143,#106144,#106145,#106146,#106147,#106148,#106149,#106150,#106151,
#106152,#106153,#106154,#106155,#106156,#106157,#106158,#106159,#106160,
#106161,#106162,#106163,#106164,#106165,#106166,#106167,#106168,#106169,
#106170,#106171,#106172,#106173,#106174,#106175,#106176,#106177,#106178,
#106179,#106180,#106181,#106182,#106183,#106184,#106185,#106186,#106187,
#106188,#106189,#106190,#106191,#106192,#106193,#106194,#106195,#106196,
#106197,#106198,#106199,#106200,#106201,#106202,#106203,#106204,#106205,
#106206,#106207,#106208,#106209,#106210,#106211,#106212,#106213,#106214,
#106215,#106216,#106217,#106218,#106219,#106220,#106221,#106222,#106223,
#106224,#106225,#106226,#106227,#106228,#106229,#106230,#106231,#106232,
#106233,#106234,#106235,#106236,#106237,#106238,#106239,#106240,#106241,
#106242,#106243,#106244,#106245,#106246,#106247),.UNSPECIFIED.,.F.,.F.,
(4,2,2,2,2,2,2,2,2,2,2,2,2,2,2,2,2,2,2,2,2,2,2,2,2,2,2,2,2,2,2,2,2,2,2,
2,2,2,2,2,2,2,2,2,2,2,2,2,2,2,2,2,2,2,2,2,2,2,2,2,2,2,2,2,2,2,2,2,2,2,2,
2,2,2,2,2,2,2,2,2,2,2,2,2,2,2,2,2,2,2,2,2,2,2,2,2,2,2,2,2,2,2,2,2,2,2,2,
2,2,2,2,2,2,2,2,2,2,2,2,2,2,2,2,2,2,2,2,2,2,2,2,2,2,2,2,4),(-2.59351319560632,
-2.58622729647481,-2.5828910286521,-2.58079840780792,-2.57886475756614,
-2.57636824993871,-2.57222640200302,-2.54442188896087,-2.50218668673736,
-2.4863039129939,-2.48078587998544,-2.47815169115976,-2.47603980137504,
-2.47481721054413,-2.47481365550069,-2.47481008690544,-2.47480650437782,
-2.47480290789427,-2.47479903883037,-2.47479510242231,-2.47479109722825,
-2.47478702163512,-2.47478287417935,-2.47477865356258,-2.47477435809535,
-2.4747699860217,-2.47476553576133,-2.47476100560858,-2.4747563936866,-2.4747516982887,
-2.47474691755708,-2.47474204951989,-2.47371676215764,-2.47234226881227,
-2.46950023768353,-2.43258570407835,-2.4009737629099,-2.38440863396358,
-2.37409713727002,-2.37084837729661,-2.36877504609808,-2.36683437516808,
-2.36429323824179,-2.3599983540294,-2.32488069726845,-2.27595609337913,
-2.26621225986546,-2.26403793530591,-2.2628029665682,-2.26172916672737,
-2.26035130298056,-2.25749226052489,-2.23432220255429,-2.19389543829676,
-2.16701319175459,-2.16080089954351,-2.15812995821089,-2.15617495824058,
-2.15437405952378,-2.15146407834257,-2.1443087833654,-2.09623415175186,
-2.05641757161317,-2.05283996628691,-2.05133047028622,-2.05023825258886,
-2.04921250722231,-2.04747019668775,-2.04274245790632,-2.00254661427086,
-1.95409223359277,-1.94848361985468,-1.94592066735513,-1.94398352098303,
-1.94215438428467,-1.93960316766758,-1.93290199156341,-1.87770481430317,
-1.8532397838111,-1.84230846741542,-1.8400580009635,-1.83880635261458,-1.83773454389397,
-1.8363804186677,-1.83424114104554,-1.82330530234437,-1.81870714839375,
-1.81437645424526,-1.76781417873323,-1.74938219701642,-1.73824679811172,
-1.73490673030146,-1.73281325542241,-1.73087985742359,-1.72838513436213,
-1.72424941044737,-1.69667985670387,-1.65436520346332,-1.63836283839693,
-1.63001370185051,-1.62794354536582,-1.6267316103303,-1.6256536018176,-1.62426148703803,
-1.62194627929144,-1.60773046460698,-1.60656384512424,-1.60507075355574,
-1.59761470273349,-1.58581497489413,-1.55294923960831,-1.53641432631062,
-1.52611631511088,-1.52286896909941,-1.52079585850479,-1.51885491497281,
-1.51631272961663,-1.51201452299214,-1.47665305033896,-1.42748800017924,
-1.41817192492958,-1.4160275905967,-1.41479917716189,-1.41372427645148,
-1.41233603847899,-1.40942413232278,-1.37758912981916,-1.33442733211732,
-1.31578836957074,-1.31205538917346,-1.30965531190433,-1.30773840874649,
-1.3055707043418,-1.3018958498089,-1.28713190177762,-1.26001648429561),
 .UNSPECIFIED.);
#1032=B_SPLINE_CURVE_WITH_KNOTS('',3,(#106253,#106254,#106255,#106256,#106257),
 .UNSPECIFIED.,.F.,.F.,(4,1,4),(82.6397395452727,82.9034253468356,82.9907454093913),
 .UNSPECIFIED.);
#1033=B_SPLINE_CURVE_WITH_KNOTS('',3,(#106258,#106259,#106260,#106261,#106262,
#106263,#106264,#106265,#106266,#106267,#106268,#106269,#106270,#106271,
#106272,#106273,#106274,#106275,#106276,#106277,#106278,#106279,#106280,
#106281,#106282,#106283,#106284,#106285,#106286,#106287,#106288,#106289,
#106290,#106291,#106292,#106293,#106294,#106295,#106296,#106297,#106298,
#106299,#106300,#106301,#106302,#106303,#106304,#106305,#106306,#106307,
#106308,#106309,#106310,#106311,#106312,#106313,#106314,#106315,#106316,
#106317,#106318,#106319,#106320,#106321,#106322,#106323,#106324,#106325,
#106326,#106327,#106328,#106329,#106330,#106331,#106332,#106333,#106334,
#106335,#106336,#106337,#106338,#106339,#106340,#106341,#106342,#106343,
#106344,#106345,#106346,#106347,#106348,#106349,#106350,#106351,#106352,
#106353,#106354,#106355,#106356,#106357,#106358,#106359,#106360,#106361,
#106362,#106363,#106364,#106365,#106366,#106367,#106368,#106369,#106370,
#106371,#106372,#106373,#106374,#106375,#106376,#106377,#106378,#106379,
#106380,#106381,#106382,#106383,#106384,#106385,#106386,#106387,#106388,
#106389,#106390,#106391,#106392,#106393,#106394,#106395,#106396,#106397,
#106398,#106399,#106400,#106401,#106402,#106403,#106404,#106405,#106406,
#106407,#106408,#106409,#106410,#106411,#106412,#106413,#106414,#106415,
#106416,#106417,#106418,#106419,#106420,#106421,#106422,#106423,#106424,
#106425,#106426,#106427,#106428,#106429,#106430,#106431,#106432,#106433,
#106434,#106435,#106436,#106437,#106438,#106439,#106440,#106441,#106442,
#106443,#106444,#106445,#106446,#106447,#106448,#106449,#106450,#106451,
#106452,#106453,#106454,#106455,#106456,#106457,#106458,#106459,#106460,
#106461,#106462,#106463,#106464,#106465,#106466,#106467,#106468,#106469,
#106470,#106471,#106472,#106473,#106474,#106475,#106476,#106477,#106478,
#106479,#106480,#106481,#106482,#106483,#106484,#106485,#106486,#106487,
#106488,#106489,#106490,#106491,#106492,#106493,#106494,#106495,#106496,
#106497,#106498,#106499,#106500,#106501,#106502,#106503,#106504,#106505,
#106506,#106507,#106508,#106509,#106510,#106511,#106512,#106513,#106514,
#106515,#106516,#106517),.UNSPECIFIED.,.F.,.F.,(4,2,2,2,2,2,2,2,2,2,2,2,
2,2,2,2,2,2,2,2,2,2,2,2,2,2,2,2,2,2,2,2,2,2,2,2,2,2,2,2,2,2,2,2,2,2,2,2,
2,2,2,2,2,2,2,2,2,2,2,2,2,2,2,2,2,2,2,2,2,2,2,2,2,2,2,2,2,2,2,2,2,2,2,2,
2,2,2,2,2,2,2,2,2,2,2,2,2,2,2,2,2,2,2,2,2,2,2,2,2,2,2,2,2,2,2,2,2,2,2,2,
2,2,2,2,2,2,2,2,2,4),(-2.66770269248702,-2.61543390608651,-2.59708901872597,
-2.58599213567297,-2.58265684473502,-2.58056483944361,-2.57863175991318,
-2.57613599181597,-2.57199537664879,-2.54419949573402,-2.50197655657685,
-2.4860982783431,-2.48058182905784,-2.47794840215327,-2.4758371254069,-2.47461489290665,
-2.47461133859609,-2.47460777046125,-2.47460418859721,-2.47460059284622,
-2.47459672452964,-2.47459278871543,-2.47458878423225,-2.4745847095446,
-2.47458056293282,-2.47457634316857,-2.47457204866205,-2.47456767749543,
-2.47456322803027,-2.47455869878193,-2.47455408788495,-2.47454939350027,
-2.47454461377057,-2.47453974666965,-2.47351462281696,-2.47214035031746,
-2.46929879256742,-2.43238860783665,-2.40078017653839,-2.38421945468437,
-2.37391039286149,-2.3706622359411,-2.36858925018365,-2.36664887490175,
-2.36410808514931,-2.35981369817105,-2.32468817729439,-2.27572965952275,
-2.26603636731641,-2.26386575406602,-2.26263172004954,-2.26155798021014,
-2.26017920818975,-2.25731488151531,-2.23382126683387,-2.22170969805593,
-2.18883046149072,-2.17227566196906,-2.16196909941451,-2.15872109813416,
-2.156648059864,-2.15470752876087,-2.15216638105854,-2.14787104409181,-2.11269116772034,
-2.06356069282311,-2.05406347989256,-2.05190645283678,-2.050675361251,-2.04960109425711,
-2.04821758978073,-2.0453293297153,-2.01983024614342,-1.97758286427438,
-1.95424053602413,-1.94848220349302,-1.94589190605637,-1.94395059511402,
-1.94212956853807,-1.9396088721162,-1.93309992710885,-1.87606425095122,
-1.85280178606955,-1.84219712827799,-1.83996667070711,-1.83871942591645,
-1.83764722297716,-1.83628724094131,-1.83412863148369,-1.82287775300273,
-1.81679515807037,-1.76734752482176,-1.74916993396683,-1.73814465114353,
-1.7348165485156,-1.73272580971532,-1.73079168593352,-1.7282914589008,-1.72413668097178,
-1.69583626693606,-1.65387892702485,-1.63817238209544,-1.62992715167251,
-1.62786559807225,-1.62665562651006,-1.62557726257417,-1.62418195649302,
-1.6218557050497,-1.607472541764,-1.60648225523406,-1.60500252507759,-1.59754601795155,
-1.58574720429294,-1.55288376098251,-1.53635000124923,-1.52605270838614,
-1.52280558884335,-1.52073262281562,-1.51879181462613,-1.51624980652628,
-1.51195189957472,-1.47659289017339,-1.42743126908458,-1.41811584365443,
-1.41597165886288,-1.41474333108927,-1.4136685053321,-1.41228036416027,
-1.40936866104105,-1.40856975518855),.UNSPECIFIED.);
#1034=B_SPLINE_CURVE_WITH_KNOTS('',3,(#106519,#106520,#106521,#106522,#106523,
#106524,#106525,#106526,#106527,#106528,#106529,#106530,#106531,#106532,
#106533,#106534,#106535,#106536,#106537,#106538,#106539,#106540,#106541,
#106542,#106543,#106544,#106545,#106546,#106547,#106548,#106549,#106550,
#106551,#106552,#106553,#106554,#106555,#106556,#106557,#106558,#106559,
#106560,#106561,#106562,#106563,#106564,#106565,#106566,#106567,#106568,
#106569,#106570,#106571,#106572,#106573,#106574,#106575,#106576,#106577,
#106578,#106579,#106580,#106581,#106582,#106583,#106584,#106585,#106586,
#106587,#106588,#106589,#106590,#106591,#106592,#106593,#106594,#106595,
#106596,#106597,#106598,#106599,#106600,#106601,#106602,#106603,#106604,
#106605,#106606,#106607,#106608,#106609,#106610,#106611,#106612,#106613,
#106614,#106615,#106616,#106617,#106618,#106619,#106620,#106621,#106622,
#106623,#106624,#106625,#106626,#106627,#106628,#106629,#106630,#106631,
#106632,#106633,#106634,#106635,#106636,#106637,#106638,#106639,#106640,
#106641,#106642,#106643,#106644,#106645,#106646,#106647,#106648,#106649,
#106650,#106651,#106652,#106653,#106654,#106655,#106656,#106657,#106658,
#106659,#106660,#106661,#106662,#106663,#106664,#106665,#106666,#106667,
#106668,#106669,#106670,#106671,#106672,#106673,#106674,#106675,#106676,
#106677,#106678,#106679,#106680,#106681,#106682,#106683,#106684,#106685,
#106686,#106687,#106688,#106689,#106690,#106691,#106692,#106693,#106694,
#106695,#106696,#106697,#106698,#106699,#106700,#106701,#106702,#106703,
#106704,#106705,#106706,#106707,#106708,#106709,#106710,#106711,#106712,
#106713,#106714,#106715,#106716,#106717,#106718,#106719,#106720,#106721,
#106722,#106723,#106724,#106725,#106726,#106727,#106728,#106729,#106730,
#106731,#106732,#106733,#106734,#106735,#106736,#106737,#106738,#106739,
#106740,#106741,#106742,#106743,#106744,#106745,#106746,#106747,#106748,
#106749,#106750,#106751,#106752,#106753,#106754,#106755,#106756,#106757,
#106758,#106759,#106760,#106761,#106762,#106763,#106764,#106765,#106766,
#106767,#106768,#106769,#106770,#106771,#106772,#106773,#106774,#106775,
#106776,#106777,#106778,#106779,#106780,#106781,#106782),.UNSPECIFIED.,
 .F.,.F.,(4,2,2,2,2,2,2,2,2,2,2,2,2,2,2,2,2,2,2,2,2,2,2,2,2,2,2,2,2,2,2,
2,2,2,2,2,2,2,2,2,2,2,2,2,2,2,2,2,2,2,2,2,2,2,2,2,2,2,2,2,2,2,2,2,2,2,2,
2,2,2,2,2,2,2,2,2,2,2,2,2,2,2,2,2,2,2,2,2,2,2,2,2,2,2,2,2,2,2,2,2,2,2,2,
2,2,2,2,2,2,2,2,2,2,2,2,2,2,2,2,2,2,2,2,2,2,2,2,2,2,2,2,4),(-1.26001648429561,
-1.25920489695078,-1.20940448836762,-1.20520124082162,-1.20354114986599,
-1.20253128660603,-1.20142696686747,-1.19985187033462,-1.19587568666747,
-1.17606163521429,-1.1471468068602,-1.10482490162242,-1.10052948659098,
-1.09798806826835,-1.09604719031824,-1.09397364468755,-1.0907245615764,
-1.08041206308618,-1.06384765514126,-1.03098457123331,-1.01705856606983,
-1.0106294555596,-0.995044836916912,-0.992443084660772,-0.991099598250274,
-0.990028480673695,-0.988768664410134,-0.986480672386839,-0.974901573923448,
-0.947909407086809,-0.896323680640296,-0.889332355187557,-0.886449723671537,
-0.884653839874391,-0.88269480875693,-0.880001167632593,-0.873656613949112,
-0.845695618422445,-0.799193315313246,-0.783080691472976,-0.780453790669127,
-0.779104905126549,-0.778033470879843,-0.776777901415799,-0.774509372324553,
-0.763271636052209,-0.737633451839069,-0.684124892294134,-0.67727192457901,
-0.674412141771313,-0.672620452228583,-0.670657920468287,-0.667944659801545,
-0.661483904869319,-0.607528601539598,-0.571346076407321,-0.568490853645776,
-0.567113737401025,-0.566040002926676,-0.564804533874532,-0.562627938470995,
-0.552851307085002,-0.503928450894076,-0.468823462713982,-0.464101471570169,
-0.46167862601721,-0.459759698495756,-0.457606763773942,-0.453997974824864,
-0.440035486926255,-0.389255795890994,-0.359425299829533,-0.356511190805702,
-0.355122608814479,-0.35404776287155,-0.35281978042695,-0.350677046768013,
-0.341381333426028,-0.322532398642188,-0.285802998947758,-0.256623995330623,
-0.252442931410543,-0.249934948227704,-0.247999556502226,-0.247958738862809,
-0.247923852040322,-0.247894029820711,-0.24786853301023,-0.247846730883511,
-0.247828085306439,-0.247805395030296,-0.247783497486897,-0.247762362612493,
-0.247741961719488,-0.247722267322392,-0.247703253072053,-0.247684893668127,
-0.247667164828339,-0.247650043226398,-0.247633506438837,-0.247617532879141,
-0.247602101991462,-0.247587193913733,-0.247572792895465,-0.247558879109898,
-0.247545433492083,-0.247532439218449,-0.247519880067256,-0.245316875653341,
-0.24143011281927,-0.236650002340525,-0.226661648557354,-0.197489855218114,
-0.149610976621307,-0.145275678286585,-0.143594266582085,-0.142580467621698,
-0.141479947671423,-0.13992389071989,-0.136065402572038,-0.117353448275053,
-0.0757357782033879,-0.0634020279927224,-0.0604358932045252,-0.0436144758865441,
-0.0399995534467219,-0.0376361158920789,-0.0357225177441432,-0.0339209984432892,
-0.0317709117344062,-0.0286342827363197,-0.000628475142166855),
 .UNSPECIFIED.);
#1035=B_SPLINE_CURVE_WITH_KNOTS('',3,(#106783,#106784,#106785,#106786,#106787,
#106788,#106789,#106790,#106791,#106792,#106793,#106794,#106795,#106796,
#106797,#106798,#106799,#106800),.UNSPECIFIED.,.F.,.F.,(4,2,2,2,2,2,2,2,
4),(-2.66758135155173,-2.62400468004738,-2.60402406129045,-2.60002990222267,
-2.59845181316381,-2.59734678412026,-2.5963373388615,-2.59468003953891,
-2.59343214472076),.UNSPECIFIED.);
#1036=B_SPLINE_CURVE_WITH_KNOTS('',3,(#106806,#106807,#106808,#106809,#106810,
#106811,#106812,#106813,#106814,#106815,#106816,#106817,#106818),
 .UNSPECIFIED.,.F.,.F.,(4,3,3,3,4),(76.3573195230834,76.458908846057,76.5605128417353,
76.6622238573892,76.7075599105292),.UNSPECIFIED.);
#1037=B_SPLINE_CURVE_WITH_KNOTS('',3,(#106819,#106820,#106821,#106822,#106823,
#106824,#106825,#106826,#106827,#106828),.UNSPECIFIED.,.F.,.F.,(4,1,1,1,
1,1,1,4),(76.7075601022117,76.9104066470643,77.9092430970262,78.9080795469881,
79.9069159969499,80.9057524469118,81.9045888968737,82.6397395452727),
 .UNSPECIFIED.);
#1038=B_SPLINE_CURVE_WITH_KNOTS('',3,(#106829,#106830,#106831,#106832,#106833,
#106834,#106835,#106836,#106837,#106838,#106839,#106840,#106841,#106842,
#106843,#106844,#106845,#106846,#106847,#106848,#106849,#106850,#106851,
#106852,#106853,#106854,#106855,#106856,#106857,#106858,#106859,#106860,
#106861,#106862,#106863,#106864,#106865,#106866,#106867,#106868,#106869,
#106870,#106871,#106872,#106873,#106874,#106875,#106876,#106877,#106878,
#106879,#106880,#106881,#106882,#106883,#106884,#106885,#106886,#106887,
#106888,#106889,#106890,#106891,#106892,#106893,#106894,#106895,#106896,
#106897,#106898,#106899,#106900,#106901,#106902,#106903,#106904,#106905,
#106906,#106907,#106908,#106909,#106910,#106911,#106912,#106913,#106914,
#106915,#106916,#106917,#106918,#106919,#106920,#106921,#106922,#106923,
#106924,#106925,#106926,#106927,#106928,#106929,#106930,#106931,#106932,
#106933,#106934,#106935,#106936,#106937,#106938,#106939,#106940,#106941,
#106942,#106943,#106944,#106945,#106946,#106947,#106948,#106949,#106950,
#106951,#106952,#106953,#106954,#106955,#106956,#106957,#106958,#106959,
#106960,#106961,#106962,#106963,#106964,#106965,#106966,#106967,#106968,
#106969,#106970,#106971,#106972,#106973,#106974,#106975,#106976,#106977,
#106978,#106979,#106980,#106981,#106982,#106983,#106984,#106985,#106986,
#106987,#106988,#106989,#106990,#106991,#106992,#106993,#106994,#106995,
#106996,#106997,#106998,#106999,#107000,#107001,#107002,#107003,#107004,
#107005,#107006,#107007,#107008,#107009,#107010,#107011,#107012,#107013,
#107014,#107015,#107016,#107017,#107018,#107019,#107020,#107021,#107022,
#107023,#107024,#107025,#107026,#107027,#107028,#107029,#107030,#107031,
#107032,#107033,#107034,#107035,#107036,#107037,#107038,#107039,#107040,
#107041,#107042,#107043,#107044,#107045,#107046,#107047,#107048,#107049,
#107050,#107051,#107052,#107053,#107054,#107055,#107056,#107057,#107058,
#107059,#107060),.UNSPECIFIED.,.F.,.F.,(4,2,2,2,2,2,2,2,2,2,2,2,2,2,2,2,
2,2,2,2,2,2,2,2,2,2,2,2,2,2,2,2,2,2,2,2,2,2,2,2,2,2,2,2,2,2,2,2,2,2,2,2,
2,2,2,2,2,2,2,2,2,2,2,2,2,2,2,2,2,2,2,2,2,2,2,2,2,2,2,2,2,2,2,2,2,2,2,2,
2,2,2,2,2,2,2,2,2,2,2,2,2,2,2,2,2,2,2,2,2,2,2,2,2,2,2,4),(-2.59343214472076,
-2.59049405177952,-2.54046226013771,-2.51631371553413,-2.50448782487539,
-2.49650821776788,-2.49356520789235,-2.4917739804419,-2.48983320130117,
-2.48729322097717,-2.48300319883559,-2.44787191663159,-2.39894810145459,
-2.38919014010936,-2.38701455334178,-2.38577915932073,-2.38470517646818,
-2.3833273220989,-2.38046913999823,-2.35760068662714,-2.31207027802872,
-2.29541852548593,-2.28506731090479,-2.28181356940159,-2.27973886362835,
-2.27779817210041,-2.27525883283369,-2.27097107139423,-2.23581092895971,
-2.18681243869875,-2.17714169331629,-2.17497209228785,-2.17373800617207,
-2.17266381785388,-2.17128394195642,-2.16906025241394,-2.15666860288048,
-2.14992522387111,-2.10271279728319,-2.08431872950774,-2.07319905836646,
-2.06986026397319,-2.06776681331326,-2.06583291058881,-2.06333679777569,
-2.05919716850347,-2.03150304958646,-1.98921351003062,-1.97327362885962,
-1.96494579070437,-1.96287710524162,-1.9616653542782,-1.96058704774786,
-1.95919394894811,-1.95687585020999,-1.94261282142306,-1.93155606646583,
-1.93131882217436,-1.89233827786464,-1.86585616222138,-1.85969294270398,
-1.8570302012477,-1.85507634752613,-1.85327309549817,-1.85035170163565,
-1.84313048537446,-1.79862196300042,-1.78473430111998,-1.76327618979293,
-1.75318371597878,-1.75098567421837,-1.74974535432619,-1.74867205301748,
-1.74730152774724,-1.74510872263625,-1.73333941156873,-1.72962683785969,
-1.72236557018538,-1.67901009148259,-1.66042268433315,-1.64921987609181,
-1.64587221396772,-1.64377679997451,-1.64184352779864,-1.63935164702255,
-1.63522643355997,-1.60809056486313,-1.56616637408107,-1.54954736726303,
-1.54098478554423,-1.53889723485167,-1.53768129588908,-1.53660390369748,
-1.5352179788294,-1.53292427248687,-1.51915032676092,-1.50784479204249,
-1.46844818147014,-1.44187537907986,-1.43570086687288,-1.43303615859763,
-1.43108195769395,-1.42927915481719,-1.4263602080251,-1.41915354398586,
-1.37307254950704,-1.33396207651879,-1.33297747694236,-1.32826979179497,
-1.32653031764444,-1.3255049915898,-1.32441216064219,-1.32290008666066,
-1.31930843287669,-1.28016623845279,-1.25968440003088),.UNSPECIFIED.);
#1039=B_SPLINE_CURVE_WITH_KNOTS('',3,(#107066,#107067,#107068,#107069,#107070,
#107071,#107072,#107073,#107074,#107075,#107076,#107077,#107078,#107079,
#107080,#107081),.UNSPECIFIED.,.F.,.F.,(4,2,2,2,2,2,2,4),(-0.0749582685536123,
-0.0267279126156495,-0.0187640072134933,-0.00802108894736205,-0.00466632906678189,
-0.00258130059291907,-0.00128118361729658,-0.000628940948285152),
 .UNSPECIFIED.);
#1040=B_SPLINE_CURVE_WITH_KNOTS('',3,(#107082,#107083,#107084,#107085,#107086,
#107087,#107088,#107089,#107090,#107091,#107092,#107093,#107094,#107095,
#107096,#107097,#107098,#107099,#107100,#107101,#107102,#107103,#107104,
#107105,#107106,#107107,#107108,#107109,#107110,#107111,#107112,#107113,
#107114,#107115,#107116,#107117,#107118,#107119,#107120,#107121,#107122,
#107123,#107124,#107125,#107126,#107127,#107128,#107129,#107130,#107131,
#107132,#107133,#107134,#107135,#107136,#107137,#107138,#107139,#107140,
#107141,#107142,#107143,#107144,#107145,#107146,#107147,#107148,#107149,
#107150,#107151,#107152,#107153,#107154,#107155,#107156,#107157,#107158,
#107159,#107160,#107161,#107162,#107163,#107164,#107165,#107166,#107167,
#107168,#107169,#107170,#107171,#107172,#107173,#107174,#107175,#107176,
#107177,#107178,#107179,#107180,#107181,#107182,#107183,#107184,#107185,
#107186,#107187,#107188,#107189,#107190,#107191,#107192,#107193,#107194,
#107195,#107196,#107197,#107198,#107199,#107200,#107201,#107202,#107203,
#107204,#107205,#107206,#107207,#107208,#107209,#107210,#107211,#107212,
#107213,#107214,#107215,#107216,#107217,#107218,#107219,#107220,#107221,
#107222,#107223,#107224,#107225,#107226,#107227,#107228,#107229,#107230,
#107231,#107232,#107233,#107234,#107235,#107236,#107237,#107238,#107239,
#107240,#107241,#107242,#107243,#107244,#107245,#107246,#107247,#107248,
#107249,#107250,#107251,#107252,#107253,#107254,#107255,#107256,#107257,
#107258,#107259,#107260,#107261,#107262),.UNSPECIFIED.,.F.,.F.,(4,3,3,3,
3,3,3,3,3,3,3,3,3,3,3,3,3,3,3,3,3,3,3,3,3,3,3,3,3,3,3,3,3,3,3,3,3,3,3,3,
3,3,3,3,3,3,3,3,3,3,3,3,3,3,3,3,3,3,3,3,4),(70.4243747954073,70.5325790413764,
70.6410991164255,70.7497863837844,70.8587740112828,70.9173879472931,71.0207826843409,
71.1240239664559,71.227143931848,71.3301985000568,71.4332217084145,71.5362475510868,
71.6393803178647,71.7425694092745,71.845941402656,71.9162243972549,72.0196191343028,
72.1228604164179,72.2259803818101,72.3290349500191,72.4320581583768,72.5350840010493,
72.6382167678274,72.7414058592372,72.8447778526189,72.9150608472168,73.0184555842648,
73.1216968663798,73.2248168317722,73.3278713999811,73.4308946083389,73.5339204510115,
73.6370532177896,73.7402423091995,73.8436143025812,73.9138972971787,74.0172920342266,
74.1205333163416,74.2236532817338,74.3267078499427,74.4297310583004,74.5327569009728,
74.6358896677508,74.7390787591606,74.8424507525422,74.9127337471406,75.0161284841885,
75.1193697663035,75.2224897316958,75.3255442999047,75.4285675082625,75.5315933509351,
75.6347261177132,75.7379152091229,75.8412872025046,75.9115701971024,76.0134810050321,
76.1152211478687,76.2168630906174,76.3184433457363,76.3573195230834),
 .UNSPECIFIED.);
#1041=B_SPLINE_CURVE_WITH_KNOTS('',3,(#107264,#107265,#107266,#107267,#107268,
#107269,#107270,#107271,#107272,#107273,#107274,#107275,#107276,#107277,
#107278,#107279,#107280,#107281,#107282,#107283,#107284,#107285,#107286,
#107287,#107288,#107289,#107290,#107291,#107292,#107293,#107294,#107295,
#107296,#107297,#107298,#107299,#107300,#107301,#107302,#107303,#107304,
#107305,#107306,#107307,#107308,#107309,#107310,#107311,#107312,#107313,
#107314,#107315,#107316,#107317,#107318,#107319,#107320,#107321,#107322,
#107323,#107324,#107325,#107326,#107327,#107328,#107329,#107330,#107331,
#107332,#107333,#107334,#107335,#107336,#107337,#107338,#107339,#107340,
#107341,#107342,#107343,#107344,#107345,#107346,#107347,#107348,#107349,
#107350,#107351,#107352,#107353,#107354,#107355,#107356,#107357,#107358,
#107359,#107360,#107361,#107362,#107363,#107364,#107365,#107366,#107367,
#107368,#107369,#107370,#107371,#107372,#107373,#107374,#107375,#107376,
#107377,#107378,#107379,#107380,#107381,#107382,#107383,#107384,#107385,
#107386,#107387,#107388,#107389,#107390,#107391,#107392,#107393,#107394,
#107395,#107396,#107397,#107398,#107399,#107400,#107401,#107402,#107403,
#107404,#107405,#107406,#107407,#107408,#107409,#107410,#107411,#107412,
#107413,#107414,#107415,#107416,#107417,#107418,#107419,#107420,#107421,
#107422,#107423,#107424,#107425,#107426,#107427,#107428,#107429,#107430,
#107431,#107432,#107433,#107434,#107435,#107436,#107437,#107438,#107439,
#107440,#107441,#107442,#107443,#107444,#107445,#107446,#107447,#107448,
#107449,#107450,#107451,#107452,#107453,#107454,#107455,#107456,#107457,
#107458,#107459,#107460,#107461,#107462,#107463,#107464,#107465,#107466,
#107467,#107468,#107469,#107470,#107471,#107472,#107473,#107474,#107475,
#107476,#107477,#107478,#107479),.UNSPECIFIED.,.F.,.F.,(4,2,2,2,2,2,2,2,
2,2,2,2,2,2,2,2,2,2,2,2,2,2,2,2,2,2,2,2,2,2,2,2,2,2,2,2,2,2,2,2,2,2,2,2,
2,2,2,2,2,2,2,2,2,2,2,2,2,2,2,2,2,2,2,2,2,2,2,2,2,2,2,2,2,2,2,2,2,2,2,2,
2,2,2,2,2,2,2,2,2,2,2,2,2,2,2,2,2,2,2,2,2,2,2,2,2,2,2,4),(-1.25968440003088,
-1.23134369063143,-1.22421241025332,-1.22130615144709,-1.21950571246795,
-1.21754976113992,-1.21487490057086,-1.20864153191671,-1.18159607626975,
-1.14087004519534,-1.11820871474527,-1.11535576177377,-1.11397896260965,
-1.11290510951051,-1.11166909066276,-1.10949053703989,-1.09968869014144,
-1.05077806094501,-1.01565732978857,-1.01136167391632,-1.00882015719558,
-1.00687922949478,-1.0048056553366,-1.00155657894078,-0.991244535246914,
-0.974681270103429,-0.94181871242264,-0.928012268689017,-0.921312713500247,
-0.905865018602465,-0.903497110758078,-0.902089531001489,-0.901009375125651,
-0.89980592473939,-0.897774117147262,-0.889883828855659,-0.875166458977492,
-0.84610353321798,-0.803698159063138,-0.799404688454027,-0.79686386219703,
-0.794923114745073,-0.792849396568352,-0.789599391503073,-0.779278469475279,
-0.762695298773928,-0.729817074534332,-0.71452118017559,-0.709793775253745,
-0.693941560887125,-0.691328748436845,-0.689982891387343,-0.688911647404452,
-0.687653730257804,-0.685374418609237,-0.673948877567028,-0.647572473611019,
-0.59512229067345,-0.588188791336395,-0.585315747071719,-0.583521640093746,
-0.581561187570464,-0.578859458459984,-0.572467088243047,-0.526046748643198,
-0.48494794489779,-0.480263095853582,-0.47852731511801,-0.477502864531078,
-0.47640986013649,-0.474895738335049,-0.47129087238757,-0.432949642134656,
-0.383317392119324,-0.376221666139646,-0.373321736379029,-0.371522742279671,
-0.369566400597489,-0.366887468622537,-0.360806601280349,-0.352445803405556,
-0.301551400708137,-0.270313240735481,-0.267401273607805,-0.266013096698057,
-0.264938280950742,-0.263710016013293,-0.26156604694954,-0.252414962827848,
-0.203666416271385,-0.167704289663162,-0.162982355730755,-0.160559557266441,
-0.158640675771371,-0.156487801866807,-0.15425804644873,-0.146612093359325,
-0.121083043180849,-0.100337614942073,-0.0610229393878702,-0.0562870044016026,
-0.0545435810105591,-0.0535177050911518,-0.0524257923617553,-0.0509174392522457,
-0.0492296204587821,-0.0462824097053656,-0.000629118990308949),
 .UNSPECIFIED.);
#1042=B_SPLINE_CURVE_WITH_KNOTS('',3,(#107480,#107481,#107482,#107483,#107484,
#107485,#107486,#107487,#107488,#107489,#107490,#107491,#107492),
 .UNSPECIFIED.,.F.,.F.,(4,3,3,3,4),(-66.6728921052185,-66.5709585796848,
-66.469095014769,-66.367250944913,-66.322858845468),.UNSPECIFIED.);
#1043=B_SPLINE_CURVE_WITH_KNOTS('',3,(#107497,#107498,#107499,#107500,#107501,
#107502,#107503,#107504,#107505,#107506,#107507,#107508,#107509,#107510,
#107511,#107512,#107513,#107514,#107515,#107516,#107517,#107518,#107519,
#107520,#107521,#107522,#107523,#107524,#107525,#107526,#107527,#107528,
#107529,#107530,#107531,#107532,#107533,#107534,#107535,#107536,#107537,
#107538,#107539,#107540,#107541,#107542,#107543,#107544,#107545,#107546,
#107547,#107548,#107549,#107550,#107551,#107552,#107553,#107554,#107555,
#107556,#107557,#107558,#107559,#107560,#107561,#107562,#107563,#107564,
#107565,#107566,#107567,#107568,#107569,#107570,#107571,#107572,#107573,
#107574,#107575,#107576,#107577,#107578,#107579,#107580,#107581,#107582,
#107583,#107584,#107585,#107586,#107587,#107588,#107589,#107590,#107591,
#107592,#107593,#107594,#107595,#107596,#107597,#107598,#107599,#107600,
#107601,#107602,#107603,#107604,#107605,#107606,#107607,#107608,#107609,
#107610,#107611,#107612,#107613,#107614,#107615,#107616,#107617,#107618,
#107619,#107620,#107621,#107622,#107623,#107624,#107625,#107626,#107627,
#107628,#107629,#107630,#107631,#107632,#107633,#107634,#107635,#107636,
#107637,#107638,#107639,#107640,#107641,#107642,#107643,#107644,#107645,
#107646,#107647,#107648,#107649,#107650,#107651,#107652,#107653,#107654,
#107655,#107656,#107657,#107658,#107659,#107660,#107661,#107662,#107663,
#107664,#107665,#107666,#107667,#107668,#107669,#107670,#107671,#107672,
#107673,#107674,#107675,#107676,#107677,#107678,#107679,#107680,#107681,
#107682,#107683,#107684,#107685,#107686,#107687,#107688,#107689,#107690,
#107691,#107692,#107693,#107694,#107695,#107696,#107697,#107698,#107699,
#107700,#107701,#107702,#107703,#107704,#107705,#107706,#107707,#107708,
#107709,#107710,#107711,#107712,#107713,#107714,#107715,#107716,#107717,
#107718,#107719,#107720,#107721,#107722,#107723,#107724,#107725,#107726,
#107727,#107728,#107729,#107730,#107731,#107732),.UNSPECIFIED.,.F.,.F.,
(4,2,2,2,2,2,2,2,2,2,2,2,2,2,2,2,2,2,2,2,2,2,2,2,2,2,2,2,2,2,2,2,2,2,2,
2,2,2,2,2,2,2,2,2,2,2,2,2,2,2,2,2,2,2,2,2,2,2,2,2,2,2,2,2,2,2,2,2,2,2,2,
2,2,2,2,2,2,2,2,2,2,2,2,2,2,2,2,2,2,2,2,2,2,2,2,2,2,2,2,2,2,2,2,2,2,2,2,
2,2,2,2,2,2,2,2,2,2,4),(-1.40860274249303,-1.39545372053415,-1.38405191255192,
-1.38177360603223,-1.38051573100286,-1.37944421601724,-1.37809762224227,
-1.37548221954635,-1.35956072507084,-1.35505839864631,-1.3344941572798,
-1.28613739827495,-1.27898801345227,-1.27607861829502,-1.27427752549132,
-1.27232188142241,-1.26964927272706,-1.26342950298786,-1.23649576466275,
-1.19596815909722,-1.1729752699172,-1.17011974512723,-1.16874239215002,
-1.16766843028723,-1.16643265125198,-1.16425539405046,-1.15447387394157,
-1.10554271681862,-1.07041410358646,-1.06611811509309,-1.06357642475794,
-1.06163537781953,-1.05956168921858,-1.05631246052951,-1.04600016133745,
-1.02943670254059,-0.996572845154755,-0.982829375741294,-0.975979431163806,
-0.975668394635018,-0.970141227948445,-0.960085624833772,-0.958003434641783,
-0.956666723725821,-0.955595910672606,-0.954330489411165,-0.952016880235014,
-0.939969961362546,-0.887892504752826,-0.85823648297296,-0.854045172676218,
-0.851534106912541,-0.849598134439495,-0.847511861535831,-0.844204716305503,
-0.833374313120382,-0.815647041064647,-0.765033835011717,-0.748652933501051,
-0.746018229818602,-0.744667621415628,-0.743596013538634,-0.742341621977587,
-0.740078712913451,-0.728939064684917,-0.703681073476061,-0.64961305370415,
-0.642806060412559,-0.639953770356868,-0.638163360840862,-0.636199471538239,
-0.633479246418707,-0.626977553308289,-0.597700080219243,-0.557147289503821,
-0.552470286680263,-0.536615849012431,-0.534003013797779,-0.532657161058179,
-0.531585928963038,-0.530328035593527,-0.52804879206617,-0.516624112560615,
-0.490250909400853,-0.437796774641233,-0.430863984088467,-0.427991076922987,
-0.426197009858696,-0.424236564324825,-0.421534777893735,-0.415141956993546,
-0.368529713838952,-0.327635551524136,-0.322942373867071,-0.321205340293311,
-0.32018065208492,-0.319087820765109,-0.317574635505883,-0.313975218995091,
-0.276193354998924,-0.225953709927059,-0.21889336642317,-0.216053366803244,
-0.21408580476914,-0.212152641387071,-0.210202118920216,-0.205222354907001,
-0.167242607375536,-0.126440833166427,-0.112446926052252,-0.110143000891382,
-0.108754236261121,-0.107676702942697,-0.106462936107806,-0.104384338263129,
-0.0959299608814828,-0.0796216983056657,-0.0749582685536123),
 .UNSPECIFIED.);
#1044=B_SPLINE_CURVE_WITH_KNOTS('',3,(#107734,#107735,#107736,#107737,#107738,
#107739,#107740,#107741,#107742,#107743,#107744,#107745,#107746,#107747,
#107748,#107749,#107750,#107751,#107752,#107753,#107754,#107755,#107756,
#107757,#107758,#107759,#107760,#107761,#107762,#107763,#107764,#107765,
#107766,#107767,#107768,#107769,#107770,#107771,#107772,#107773,#107774,
#107775,#107776,#107777,#107778,#107779,#107780,#107781,#107782,#107783,
#107784,#107785,#107786,#107787,#107788,#107789,#107790,#107791,#107792,
#107793,#107794,#107795,#107796,#107797,#107798,#107799,#107800,#107801,
#107802,#107803,#107804,#107805,#107806,#107807,#107808,#107809,#107810,
#107811,#107812,#107813,#107814,#107815,#107816,#107817,#107818,#107819,
#107820,#107821,#107822,#107823,#107824,#107825,#107826,#107827,#107828,
#107829,#107830,#107831,#107832,#107833,#107834,#107835,#107836,#107837,
#107838,#107839,#107840,#107841,#107842,#107843,#107844,#107845,#107846,
#107847,#107848,#107849,#107850,#107851,#107852,#107853,#107854,#107855,
#107856,#107857,#107858,#107859,#107860,#107861,#107862,#107863,#107864,
#107865,#107866,#107867,#107868,#107869,#107870,#107871,#107872,#107873,
#107874,#107875,#107876,#107877,#107878,#107879,#107880,#107881,#107882,
#107883,#107884,#107885,#107886,#107887,#107888,#107889,#107890,#107891,
#107892,#107893,#107894,#107895,#107896,#107897,#107898,#107899,#107900,
#107901,#107902,#107903,#107904,#107905,#107906,#107907,#107908,#107909,
#107910,#107911),.UNSPECIFIED.,.F.,.F.,(4,3,3,3,3,3,3,3,3,3,3,3,3,3,3,3,
3,3,3,3,3,3,3,3,3,3,3,3,3,3,3,3,3,3,3,3,3,3,3,3,3,3,3,3,3,3,3,3,3,3,3,3,
3,3,3,3,3,3,3,4),(-66.322858845468,-66.2209269943692,-66.1189509138928,
-66.0167874984565,-65.9232056974837,-65.8198109604357,-65.7165696783207,
-65.6134497129284,-65.5103951447195,-65.4073719363617,-65.3043460936892,
-65.201213326911,-65.0980242355013,-64.9946522421195,-64.9243692475218,
-64.8209745104739,-64.7177332283589,-64.6146132629666,-64.5115586947577,
-64.4085354864,-64.3055096437274,-64.2023768769493,-64.0991877855396,-63.9958157921579,
-63.9255327975599,-63.822138060512,-63.718896778397,-63.6157768130047,-63.5127222447958,
-63.4096990364381,-63.3066731937654,-63.2035404269873,-63.1003513355775,
-62.9969793421958,-62.9266963475981,-62.8233016105501,-62.7200603284354,
-62.6169403630431,-62.5138857948342,-62.4108625864764,-62.3078367438042,
-62.2047039770261,-62.1015148856164,-61.9981428922348,-61.9278598976362,
-61.8244651605882,-61.7212238784728,-61.6181039130805,-61.5150493448716,
-61.4120261365139,-61.3090002938414,-61.2058675270632,-61.1026784356534,
-60.9993064422717,-60.9290234476743,-60.8220651862384,-60.7139755891885,
-60.6074364851718,-60.4985716416054,-60.3897067980389),.UNSPECIFIED.);
#1045=B_SPLINE_CURVE_WITH_KNOTS('',3,(#107912,#107913,#107914,#107915),
 .UNSPECIFIED.,.F.,.F.,(4,4),(-60.389703770172,-60.0402340848269),
 .UNSPECIFIED.);
#1046=B_SPLINE_CURVE_WITH_KNOTS('',3,(#107921,#107922,#107923,#107924,#107925,
#107926),.UNSPECIFIED.,.F.,.F.,(4,2,4),(-0.075040891899263,-0.0536888394344463,
-0.000629601840572249),.UNSPECIFIED.);
#1047=B_SPLINE_CURVE_WITH_KNOTS('',3,(#107927,#107928,#107929,#107930,#107931,
#107932,#107933,#107934,#107935,#107936,#107937,#107938,#107939,#107940,
#107941,#107942,#107943,#107944,#107945,#107946,#107947,#107948,#107949,
#107950,#107951,#107952,#107953,#107954,#107955,#107956,#107957,#107958,
#107959,#107960,#107961,#107962,#107963,#107964,#107965,#107966,#107967,
#107968,#107969,#107970,#107971,#107972,#107973,#107974,#107975,#107976,
#107977,#107978,#107979,#107980,#107981,#107982,#107983,#107984,#107985,
#107986,#107987,#107988,#107989,#107990,#107991,#107992,#107993,#107994,
#107995,#107996,#107997,#107998,#107999,#108000,#108001,#108002,#108003,
#108004,#108005,#108006,#108007,#108008,#108009,#108010,#108011,#108012,
#108013,#108014,#108015,#108016,#108017,#108018,#108019,#108020,#108021,
#108022,#108023,#108024,#108025,#108026,#108027,#108028,#108029,#108030,
#108031,#108032,#108033,#108034,#108035,#108036,#108037,#108038,#108039,
#108040,#108041,#108042,#108043,#108044,#108045,#108046,#108047,#108048,
#108049,#108050,#108051,#108052,#108053,#108054,#108055,#108056,#108057,
#108058,#108059,#108060,#108061,#108062,#108063,#108064,#108065,#108066,
#108067,#108068,#108069,#108070,#108071,#108072,#108073,#108074,#108075,
#108076,#108077,#108078,#108079,#108080,#108081,#108082,#108083,#108084,
#108085,#108086,#108087,#108088,#108089,#108090,#108091,#108092,#108093,
#108094,#108095,#108096,#108097,#108098,#108099,#108100,#108101,#108102,
#108103,#108104,#108105,#108106,#108107,#108108,#108109,#108110,#108111,
#108112,#108113,#108114,#108115,#108116,#108117,#108118,#108119,#108120,
#108121,#108122,#108123,#108124,#108125,#108126,#108127,#108128,#108129,
#108130,#108131,#108132,#108133,#108134,#108135,#108136,#108137,#108138,
#108139,#108140,#108141,#108142,#108143,#108144,#108145,#108146,#108147,
#108148,#108149,#108150,#108151,#108152,#108153,#108154,#108155,#108156,
#108157,#108158,#108159,#108160,#108161,#108162,#108163,#108164,#108165,
#108166,#108167,#108168,#108169,#108170,#108171,#108172,#108173,#108174,
#108175,#108176,#108177,#108178),.UNSPECIFIED.,.F.,.F.,(4,2,2,2,2,2,2,2,
2,2,2,2,2,2,2,2,2,2,2,2,2,2,2,2,2,2,2,2,2,2,2,2,2,2,2,2,2,2,2,2,2,2,2,2,
2,2,2,2,2,2,2,2,2,2,2,2,2,2,2,2,2,2,2,2,2,2,2,2,2,2,2,2,2,2,2,2,2,2,2,2,
2,2,2,2,2,2,2,2,2,2,2,2,2,2,2,2,2,2,2,2,2,2,2,2,2,2,2,2,2,2,2,2,2,2,2,2,
2,2,2,2,2,2,2,2,2,4),(-2.66807656983836,-2.66001931216341,-2.65566187021585,
-2.65424879941531,-2.65318148796654,-2.65215122106027,-2.65097124285194,
-2.64904592064653,-2.64298004572499,-2.64169796462927,-2.63389713220412,
-2.58067129022967,-2.56294088045462,-2.55210929912035,-2.54880138677269,
-2.54671454326925,-2.5447779822075,-2.54226607056276,-2.53807319770196,
-2.50861277988315,-2.46747060755929,-2.45202922886731,-2.44661324534596,
-2.44401378375114,-2.44190666294874,-2.44069382405631,-2.44069071036685,
-2.44068757765006,-2.4406844262157,-2.44068125547413,-2.44067806521928,
-2.44067485554611,-2.44067162617671,-2.44066837713124,-2.44066510804369,
-2.440661818944,-2.44065850972164,-2.44065518013926,-2.44065184303295,-2.44064849146409,
-2.4406451186021,-2.44064172430211,-2.4406382977067,-2.43961003975432,-2.43822996682275,
-2.43536006662262,-2.40000187929051,-2.36702700814441,-2.34413886403262,
-2.33844071610385,-2.33586108299189,-2.33392114450774,-2.33209656636895,
-2.32956323339432,-2.32297765799664,-2.26661514864444,-2.24290774166351,
-2.23218005588033,-2.22994169397189,-2.22869257256167,-2.22762033104054,
-2.22626232395855,-2.22411065702757,-2.21297838061014,-2.16172584551341,
-2.13312487315829,-2.12670359206788,-2.12399675560698,-2.1220351859839,
-2.1202418436328,-2.11737390656077,-2.11047278086461,-2.05759631778182,
-2.03154060316174,-2.02019487474647,-2.01791993584475,-2.01666286978899,
-2.01559140711415,-2.01424406876241,-2.01162484057531,-1.99562716149847,
-1.99011655002598,-1.97569213356159,-1.94279678023562,-1.92622947076308,
-1.91591640674569,-1.91266704127572,-1.91059329681986,-1.90865222022573,
-1.90611052492405,-1.9018146360312,-1.86668065146954,-1.81771775944691,
-1.80800519245818,-1.80583270591349,-1.80459798537159,-1.80352389101702,
-1.80214498157591,-1.79928146642341,-1.76328492711041,-1.73052088549797,
-1.70797122228241,-1.70231844785027,-1.69974697700491,-1.69780814426694,
-1.69598091063723,-1.69343796585279,-1.68679253526116,-1.63099604229814,
-1.59810930967717,-1.59456242182821,-1.59305797213324,-1.59196642319294,
-1.59093892317369,-1.58918851509386,-1.5844091556551,-1.547236227462,-1.496959549346,
-1.49055691298743,-1.4878530639403,-1.48589188443366,-1.4840976754684,-1.48122568543685,
-1.47430099954898,-1.42172907120572,-1.40860274249303),.UNSPECIFIED.);
#1048=B_SPLINE_CURVE_WITH_KNOTS('',3,(#108180,#108181,#108182,#108183,#108184,
#108185,#108186,#108187,#108188,#108189),.UNSPECIFIED.,.F.,.F.,(4,1,1,1,
1,1,1,4),(-60.0402340848269,-59.9301869977125,-58.9313505477506,-57.9325140977887,
-56.9336776478268,-55.934841197865,-54.9360047479031,-54.1065275202913),
 .UNSPECIFIED.);
#1049=B_SPLINE_CURVE_WITH_KNOTS('',3,(#108190,#108191,#108192,#108193,#108194,
#108195,#108196,#108197,#108198,#108199,#108200,#108201,#108202,#108203,
#108204,#108205,#108206,#108207,#108208,#108209,#108210,#108211),
 .UNSPECIFIED.,.F.,.F.,(4,2,2,2,2,2,2,2,2,2,4),(-2.66761363830502,-2.64338362104628,
-2.63625165986871,-2.63446074350259,-2.63324577351584,-2.63223669094568,
-2.63116210710082,-2.62977606482891,-2.62687504598501,-2.59995451275591,
-2.59351250887444),.UNSPECIFIED.);
#1050=B_SPLINE_CURVE_WITH_KNOTS('',3,(#108216,#108217,#108218,#108219,#108220,
#108221,#108222,#108223,#108224,#108225,#108226,#108227,#108228,#108229,
#108230,#108231,#108232,#108233,#108234,#108235,#108236,#108237,#108238,
#108239,#108240,#108241,#108242,#108243,#108244,#108245,#108246,#108247,
#108248,#108249,#108250,#108251,#108252,#108253,#108254,#108255,#108256,
#108257,#108258,#108259,#108260,#108261,#108262,#108263,#108264,#108265,
#108266,#108267,#108268,#108269,#108270,#108271,#108272,#108273,#108274,
#108275,#108276,#108277,#108278,#108279,#108280,#108281,#108282,#108283,
#108284,#108285,#108286,#108287,#108288,#108289,#108290,#108291,#108292,
#108293,#108294,#108295,#108296,#108297,#108298,#108299,#108300,#108301,
#108302,#108303,#108304,#108305,#108306,#108307,#108308,#108309,#108310,
#108311,#108312,#108313,#108314,#108315,#108316,#108317,#108318,#108319,
#108320,#108321,#108322,#108323,#108324,#108325,#108326,#108327,#108328,
#108329,#108330,#108331,#108332,#108333,#108334,#108335,#108336,#108337,
#108338,#108339,#108340,#108341,#108342,#108343,#108344,#108345,#108346,
#108347,#108348,#108349,#108350,#108351,#108352,#108353,#108354,#108355,
#108356,#108357,#108358,#108359,#108360,#108361,#108362,#108363,#108364,
#108365,#108366,#108367,#108368,#108369,#108370,#108371,#108372,#108373,
#108374,#108375,#108376,#108377,#108378,#108379,#108380,#108381,#108382,
#108383,#108384,#108385,#108386,#108387,#108388,#108389,#108390,#108391,
#108392,#108393,#108394,#108395,#108396,#108397,#108398,#108399,#108400,
#108401,#108402,#108403,#108404,#108405,#108406,#108407,#108408,#108409,
#108410,#108411,#108412,#108413,#108414,#108415,#108416,#108417,#108418,
#108419,#108420,#108421,#108422,#108423,#108424,#108425,#108426,#108427,
#108428,#108429,#108430,#108431,#108432,#108433,#108434,#108435,#108436,
#108437,#108438,#108439,#108440,#108441,#108442,#108443,#108444,#108445,
#108446,#108447,#108448,#108449,#108450,#108451,#108452,#108453,#108454,
#108455,#108456,#108457),.UNSPECIFIED.,.F.,.F.,(4,2,2,2,2,2,2,2,2,2,2,2,
2,2,2,2,2,2,2,2,2,2,2,2,2,2,2,2,2,2,2,2,2,2,2,2,2,2,2,2,2,2,2,2,2,2,2,2,
2,2,2,2,2,2,2,2,2,2,2,2,2,2,2,2,2,2,2,2,2,2,2,2,2,2,2,2,2,2,2,2,2,2,2,2,
2,2,2,2,2,2,2,2,2,2,2,2,2,2,2,2,2,2,2,2,2,2,2,2,2,2,2,2,2,2,2,2,2,2,2,2,
4),(-1.4083648719342,-1.38228065803757,-1.36894127842204,-1.36538644960133,
-1.36324542445129,-1.36132425816373,-1.35888107498145,-1.35500675348651,
-1.33393386252568,-1.27612144912632,-1.26116153864079,-1.25881363304285,
-1.25741190086447,-1.25633256740672,-1.25512596347766,-1.25307993708088,
-1.24502288644303,-1.22984433276336,-1.1899497876185,-1.15890724031151,
-1.15468587745723,-1.15216604826746,-1.15022871693044,-1.14814628849906,
-1.14485652896388,-1.13418333782302,-1.11681271534813,-1.06811113144221,
-1.0615961970822,-1.04897429092784,-1.04673866878302,-1.04535530922547,
-1.04428092999729,-1.04304946623855,-1.0408911972377,-1.03137945064811,
-0.982228280512713,-0.947034266730386,-0.942738120907567,-0.940196620859603,
-0.938255882409529,-0.936182681563432,-0.932934547373618,-0.922628505026184,
-0.906077741869524,-0.873227896211311,-0.860310720820461,-0.837608632169213,
-0.834755202051013,-0.833378495829121,-0.832304867256694,-0.831069278578373,
-0.828891894387172,-0.81910213692217,-0.770194401526692,-0.735078970921858,
-0.730784261169856,-0.728243315161181,-0.726302829608377,-0.724229733925277,
-0.720981420008596,-0.710671903867421,-0.694112800822422,-0.661258068670178,
-0.647484848121893,-0.64071664199297,-0.639061302700117,-0.625189382805616,
-0.622889893585463,-0.621502516926235,-0.620425264313628,-0.619210919235713,
-0.617129322019864,-0.608635437510486,-0.592211559054857,-0.550103913138771,
-0.522873976770003,-0.518747325349785,-0.516255509253578,-0.514322830978031,
-0.512228603140846,-0.508884011407604,-0.497702379996471,-0.479164179919319,
-0.434965958872584,-0.413688344646884,-0.410871718878125,-0.409502370161695,
-0.408429535609674,-0.407189246296834,-0.40499001083307,-0.394870774261701,
-0.373313283791549,-0.363916869376676,-0.31488853818834,-0.307769058459617,
-0.304865435229307,-0.303065968954601,-0.301110552577836,-0.298435483067391,
-0.29219732858794,-0.265103892615965,-0.225442438814623,-0.201826409179347,
-0.198964970216695,-0.197586822993611,-0.19655964682314,-0.195366835491709,
-0.1933863944972,-0.190950416575893,-0.186002759025304,-0.172495020457729,
-0.150027583419131,-0.10305833797812,-0.095871369505978,-0.0929564727872435,
-0.0911549606563658,-0.0892012124947926,-0.086535416674339,-0.0803506587845703,
-0.075040891899263),.UNSPECIFIED.);
#1051=B_SPLINE_CURVE_WITH_KNOTS('',3,(#108458,#108459,#108460,#108461,#108462,
#108463,#108464,#108465,#108466,#108467,#108468,#108469,#108470,#108471,
#108472,#108473,#108474,#108475,#108476,#108477,#108478,#108479,#108480,
#108481,#108482,#108483,#108484,#108485,#108486,#108487,#108488,#108489,
#108490,#108491,#108492,#108493,#108494,#108495,#108496,#108497,#108498,
#108499,#108500,#108501,#108502,#108503,#108504,#108505,#108506,#108507,
#108508,#108509,#108510,#108511,#108512,#108513,#108514,#108515,#108516,
#108517,#108518,#108519,#108520,#108521,#108522,#108523,#108524,#108525,
#108526,#108527,#108528,#108529,#108530,#108531,#108532,#108533,#108534,
#108535,#108536,#108537,#108538,#108539,#108540,#108541,#108542,#108543,
#108544,#108545,#108546,#108547,#108548,#108549,#108550,#108551,#108552,
#108553,#108554,#108555,#108556,#108557,#108558,#108559,#108560,#108561,
#108562,#108563,#108564,#108565,#108566,#108567,#108568,#108569,#108570,
#108571,#108572,#108573,#108574,#108575,#108576,#108577,#108578,#108579,
#108580,#108581,#108582,#108583,#108584,#108585,#108586,#108587,#108588,
#108589,#108590,#108591,#108592,#108593,#108594,#108595,#108596,#108597,
#108598,#108599,#108600,#108601,#108602,#108603,#108604,#108605,#108606,
#108607,#108608,#108609,#108610,#108611,#108612,#108613,#108614,#108615,
#108616,#108617,#108618,#108619,#108620,#108621,#108622,#108623,#108624,
#108625,#108626,#108627,#108628,#108629,#108630,#108631,#108632,#108633,
#108634,#108635,#108636,#108637,#108638,#108639,#108640,#108641,#108642,
#108643,#108644,#108645,#108646,#108647,#108648,#108649,#108650,#108651,
#108652,#108653,#108654,#108655,#108656,#108657,#108658,#108659,#108660,
#108661,#108662,#108663,#108664,#108665,#108666,#108667,#108668,#108669,
#108670,#108671,#108672,#108673,#108674,#108675,#108676,#108677,#108678,
#108679,#108680,#108681,#108682,#108683,#108684,#108685),.UNSPECIFIED.,
 .F.,.F.,(4,2,2,2,2,2,2,2,2,2,2,2,2,2,2,2,2,2,2,2,2,2,2,2,2,2,2,2,2,2,2,
2,2,2,2,2,2,2,2,2,2,2,2,2,2,2,2,2,2,2,2,2,2,2,2,2,2,2,2,2,2,2,2,2,2,2,2,
2,2,2,2,2,2,2,2,2,2,2,2,2,2,2,2,2,2,2,2,2,2,2,2,2,2,2,2,2,2,2,2,2,2,2,2,
2,2,2,2,2,2,2,2,2,2,4),(-2.59351250887444,-2.58627132755899,-2.57475056578942,
-2.54617420876759,-2.5322760739487,-2.52867254583601,-2.5265206756222,-2.52460139815959,
-2.52217635843806,-2.51744459412592,-2.4800073394474,-2.42965592482369,
-2.42318153346149,-2.42129005227563,-2.42027907783809,-2.41920580512948,
-2.41783413989595,-2.41563725140815,-2.40380161873765,-2.34640696934181,
-2.32984084338238,-2.31952895204551,-2.31628018793202,-2.31420688296764,
-2.31226625687532,-2.30972520792143,-2.30543053797334,-2.27032333094732,
-2.22142962689166,-2.21165056862751,-2.20947386375746,-2.20823838682896,
-2.20716468515013,-2.20578765320441,-2.20293276527677,-2.16673537944714,
-2.13404718358941,-2.11160908086825,-2.10597201544872,-2.10340378344222,
-2.10146579932734,-2.09963819310631,-2.09709284592049,-2.09042983160154,
-2.03483734684125,-2.01063326760602,-1.99977167645199,-1.99752536847757,
-1.99627460970123,-1.99520268683062,-1.99384729454306,-1.99119018487353,
-1.97422692051994,-1.92398177534601,-1.90639237712722,-1.89562381061545,
-1.89232356372019,-1.89023888066884,-1.88830247942656,-1.8857881596038,
-1.88158552044819,-1.85136840109467,-1.79985871250863,-1.7878695760094,
-1.78555922765983,-1.78429457785566,-1.78322381824376,-1.78188641330958,
-1.77980174823529,-1.76970861435776,-1.76421760799779,-1.75679086914864,
-1.74328321183606,-1.71040117781003,-1.69384733664869,-1.6835406779019,
-1.68029227752141,-1.67821889588199,-1.67627798108125,-1.67373624105447,
-1.66943970141705,-1.63422230022242,-1.58497685489194,-1.57559915198036,
-1.5734503440178,-1.57222092170071,-1.57114614916315,-1.56975940908192,
-1.56751266758141,-1.55467956074227,-1.55251360106794,-1.50523272241264,
-1.47670828858993,-1.47029625899942,-1.46759104624969,-1.46562982511807,
-1.46383623091739,-1.46096664820263,-1.45405512645051,-1.4013235146106,
-1.37516890081238,-1.36379827027713,-1.36152196775808,-1.36026463393816,
-1.35919323748336,-1.3578463569948,-1.35522911889583,-1.33926696600732,
-1.33432291560366,-1.32867693141128,-1.28171657000092,-1.28027319717024,
-1.26123204158777,-1.25985393253769),.UNSPECIFIED.);
#1052=B_SPLINE_CURVE_WITH_KNOTS('',3,(#108691,#108692,#108693,#108694,#108695,
#108696,#108697,#108698,#108699,#108700,#108701,#108702,#108703,#108704,
#108705,#108706),.UNSPECIFIED.,.F.,.F.,(4,2,2,2,2,2,2,4),(-0.0747637516645625,
-0.0741311798278147,-0.0730589563255482,-0.0718129938420133,-0.069588043911114,
-0.0590694513428154,-0.0361125965627976,-0.000629543915810415),
 .UNSPECIFIED.);
#1053=B_SPLINE_CURVE_WITH_KNOTS('',3,(#108707,#108708,#108709,#108710,#108711,
#108712,#108713,#108714,#108715,#108716,#108717,#108718,#108719,#108720,
#108721,#108722,#108723,#108724,#108725,#108726,#108727,#108728,#108729,
#108730,#108731,#108732,#108733,#108734,#108735,#108736,#108737,#108738,
#108739,#108740,#108741,#108742,#108743,#108744,#108745,#108746,#108747,
#108748,#108749,#108750,#108751,#108752,#108753,#108754,#108755,#108756,
#108757,#108758,#108759,#108760,#108761,#108762,#108763,#108764,#108765,
#108766,#108767,#108768,#108769,#108770,#108771,#108772,#108773,#108774,
#108775,#108776,#108777,#108778,#108779,#108780,#108781,#108782,#108783,
#108784,#108785,#108786,#108787,#108788,#108789,#108790,#108791,#108792,
#108793,#108794,#108795,#108796,#108797,#108798,#108799,#108800,#108801,
#108802,#108803,#108804,#108805,#108806,#108807,#108808,#108809,#108810,
#108811,#108812,#108813,#108814,#108815,#108816,#108817,#108818,#108819,
#108820,#108821,#108822,#108823,#108824,#108825,#108826,#108827,#108828,
#108829,#108830,#108831,#108832,#108833,#108834,#108835,#108836,#108837,
#108838,#108839,#108840,#108841,#108842,#108843,#108844,#108845,#108846,
#108847,#108848,#108849,#108850,#108851,#108852,#108853,#108854,#108855,
#108856,#108857,#108858,#108859,#108860,#108861,#108862,#108863,#108864,
#108865,#108866,#108867,#108868,#108869,#108870,#108871,#108872,#108873,
#108874,#108875,#108876,#108877,#108878,#108879,#108880,#108881,#108882,
#108883,#108884,#108885,#108886,#108887,#108888,#108889,#108890,#108891,
#108892,#108893,#108894,#108895,#108896,#108897,#108898,#108899,#108900,
#108901,#108902,#108903,#108904,#108905,#108906,#108907,#108908,#108909,
#108910,#108911,#108912,#108913,#108914,#108915,#108916,#108917,#108918,
#108919,#108920,#108921,#108922,#108923,#108924,#108925,#108926,#108927,
#108928,#108929,#108930),.UNSPECIFIED.,.F.,.F.,(4,2,2,2,2,2,2,2,2,2,2,2,
2,2,2,2,2,2,2,2,2,2,2,2,2,2,2,2,2,2,2,2,2,2,2,2,2,2,2,2,2,2,2,2,2,2,2,2,
2,2,2,2,2,2,2,2,2,2,2,2,2,2,2,2,2,2,2,2,2,2,2,2,2,2,2,2,2,2,2,2,2,2,2,2,
2,2,2,2,2,2,2,2,2,2,2,2,2,2,2,2,2,2,2,2,2,2,2,2,2,2,2,4),(-2.66759551301063,
-2.64226750593368,-2.63914030665614,-2.63699407964818,-2.63519314844083,
-2.63327906761791,-2.63090974149732,-2.62727593515308,-2.61016939536854,
-2.59797798888022,-2.56928353171966,-2.54370956853474,-2.5324883834596,
-2.53022107940407,-2.52896588673696,-2.52789459429043,-2.52654565169851,
-2.52391794688924,-2.50779178616906,-2.50379742664539,-2.45804564367148,
-2.43957118040182,-2.43218401642221,-2.42665861840623,-2.42412186227216,
-2.42229832814302,-2.4204978465425,-2.41758902621197,-2.41043901546901,
-2.36229640204076,-2.32255563283699,-2.31897892562159,-2.31746972719541,
-2.3163776943593,-2.31535209834435,-2.31360998963901,-2.30888249688065,
-2.26870167715171,-2.22139730934245,-2.21500291564738,-2.21230110696522,
-2.21034088207934,-2.20854718415339,-2.20567522142932,-2.19874651514277,
-2.14629595725478,-2.11995998655112,-2.10854480352007,-2.10626638520139,
-2.10500878977185,-2.10393771956789,-2.10259194741275,-2.09997891037995,
-2.08410713777049,-2.07939135327073,-2.06407848434781,-2.03118220844407,
-2.01460696166349,-2.00429114530251,-2.00104207632652,-1.99896880056252,
-1.99702835894149,-1.99448777821134,-1.99019440755108,-1.9551640810914,
-1.90649186167509,-1.89645175727684,-1.89425760298284,-1.89301834784435,
-1.89194525309181,-1.890574062135,-1.88837840748431,-1.87655871576081,-1.87290461442835,
-1.87267890003012,-1.8658133562767,-1.85208116146166,-1.81920064391645,
-1.80264597048692,-1.79233926071727,-1.78909109291391,-1.78701791948844,
-1.78507724158568,-1.78253587237868,-1.77824009539095,-1.74304764195883,
-1.69387979804871,-1.68442083645631,-1.68226640823787,-1.68103583442675,
-1.67996139388663,-1.67857684341219,-1.6756835246681,-1.6496508754464,-1.61148605333721,
-1.58245989248429,-1.57806455212859,-1.57574112333995,-1.57382963546072,
-1.57160564939747,-1.56777763010058,-1.5527172196965,-1.50055201496992,
-1.48170759679173,-1.47241233146421,-1.47026956557208,-1.46904153158635,
-1.4679666243447,-1.46657793108343,-1.46366349277898,-1.43361917560424,
-1.4083648719342),.UNSPECIFIED.);
#1054=B_SPLINE_CURVE_WITH_KNOTS('',3,(#108932,#108933,#108934,#108935,#108936,
#108937,#108938,#108939,#108940,#108941,#108942,#108943,#108944,#108945,
#108946,#108947,#108948,#108949,#108950,#108951,#108952,#108953,#108954,
#108955,#108956,#108957,#108958,#108959,#108960,#108961,#108962,#108963,
#108964,#108965,#108966,#108967,#108968,#108969,#108970,#108971,#108972,
#108973,#108974,#108975,#108976,#108977,#108978,#108979,#108980,#108981,
#108982,#108983,#108984,#108985,#108986,#108987,#108988,#108989,#108990,
#108991,#108992,#108993,#108994,#108995,#108996,#108997,#108998,#108999,
#109000,#109001,#109002,#109003,#109004,#109005,#109006,#109007,#109008,
#109009,#109010,#109011,#109012,#109013,#109014,#109015,#109016,#109017,
#109018,#109019,#109020,#109021,#109022,#109023,#109024,#109025,#109026,
#109027,#109028,#109029,#109030,#109031,#109032,#109033,#109034,#109035,
#109036,#109037,#109038,#109039,#109040,#109041,#109042,#109043,#109044,
#109045,#109046,#109047,#109048,#109049,#109050,#109051,#109052,#109053,
#109054,#109055,#109056,#109057,#109058,#109059,#109060,#109061,#109062,
#109063,#109064,#109065,#109066,#109067,#109068,#109069,#109070,#109071,
#109072,#109073,#109074,#109075,#109076,#109077,#109078,#109079,#109080,
#109081,#109082,#109083,#109084,#109085,#109086,#109087,#109088,#109089,
#109090,#109091,#109092,#109093,#109094,#109095,#109096,#109097,#109098,
#109099,#109100,#109101,#109102,#109103,#109104,#109105,#109106,#109107,
#109108,#109109,#109110,#109111,#109112,#109113,#109114,#109115,#109116,
#109117,#109118,#109119,#109120,#109121,#109122,#109123,#109124,#109125,
#109126,#109127,#109128,#109129,#109130,#109131,#109132,#109133,#109134,
#109135,#109136,#109137,#109138,#109139,#109140,#109141),.UNSPECIFIED.,
 .F.,.F.,(4,2,2,2,2,2,2,2,2,2,2,2,2,2,2,2,2,2,2,2,2,2,2,2,2,2,2,2,2,2,2,
2,2,2,2,2,2,2,2,2,2,2,2,2,2,2,2,2,2,2,2,2,2,2,2,2,2,2,2,2,2,2,2,2,2,2,2,
2,2,2,2,2,2,2,2,2,2,2,2,2,2,2,2,2,2,2,2,2,2,2,2,2,2,2,2,2,2,2,2,2,2,2,2,
2,4),(-1.25985393253769,-1.25747070720351,-1.25506188878625,-1.25314411303961,
-1.25098192113377,-1.24733218977863,-1.23288110106248,-1.1824923785715,
-1.15282398413172,-1.14990946594436,-1.14852068833715,-1.14744569067698,
-1.14621753456537,-1.14407449709132,-1.13477745367465,-1.11592580221188,
-1.07547219421632,-1.06319339210751,-1.04861346996789,-1.04482746231387,
-1.0426129887951,-1.04070068330876,-1.03836497855085,-1.03391186143486,
-1.00287554189128,-0.954897516395568,-0.940308393613797,-0.937976016854732,
-0.936578767727052,-0.935499963058658,-0.934290692063161,-0.932232960337385,
-0.924037466166763,-0.908471121932689,-0.866887193211196,-0.83798284483716,
-0.833811357428992,-0.831306000739872,-0.829370800318638,-0.827281764971649,
-0.823962535307346,-0.813022830397436,-0.795046075348513,-0.744623015337069,
-0.728417150603735,-0.725789275347843,-0.724440079623504,-0.723368498715762,
-0.722112872809143,-0.719844534118631,-0.70861366263376,-0.683004469102693,
-0.629442223705916,-0.622592174645762,-0.619732650444161,-0.617940844231113,
-0.615977959971502,-0.613263798639319,-0.606798928859718,-0.552723562412723,
-0.516660360537288,-0.513800649203694,-0.512422547116781,-0.51134859757237,
-0.510113505817779,-0.507939068487506,-0.498196788353505,-0.449237575063062,
-0.414102805498129,-0.409806352309035,-0.407264642758628,-0.405323728394954,
-0.403250324181468,-0.400001839122923,-0.389694411770858,-0.373141166049173,
-0.340287485000375,-0.327284836256106,-0.304664024465874,-0.301812373959264,
-0.30043594147997,-0.299362251126977,-0.298126280334976,-0.295947477759373,
-0.286138962867638,-0.237241698828617,-0.202131567173052,-0.197834504628224,
-0.195292756173294,-0.193351997241082,-0.191344263162471,-0.188242470093938,
-0.184615851054495,-0.177819649992327,-0.161438223436073,-0.128729467479277,
-0.0927003709452161,-0.0898402865255275,-0.0884622746523991,-0.0873885221057937,
-0.086153799858813,-0.0839803544989066,-0.0742481400092202,-0.0252918468826534,
-0.000629465204745831),.UNSPECIFIED.);
#1055=B_SPLINE_CURVE_WITH_KNOTS('',3,(#109142,#109143,#109144,#109145,#109146,
#109147,#109148,#109149,#109150,#109151,#109152,#109153,#109154,#109155,
#109156,#109157,#109158,#109159,#109160,#109161,#109162,#109163),
 .UNSPECIFIED.,.F.,.F.,(4,2,2,2,2,2,2,2,2,2,4),(-2.66786964950218,-2.66007560444753,
-2.65477901912715,-2.65233557188793,-2.65045366453286,-2.64861290556403,
-2.64678645097458,-2.644245988198,-2.63905467741707,-2.62654410744952,-2.59345435029626),
 .UNSPECIFIED.);
#1056=B_SPLINE_CURVE_WITH_KNOTS('',3,(#109168,#109169,#109170,#109171,#109172,
#109173,#109174,#109175,#109176,#109177,#109178,#109179,#109180,#109181,
#109182,#109183,#109184,#109185,#109186,#109187,#109188,#109189,#109190,
#109191,#109192,#109193,#109194,#109195,#109196,#109197,#109198,#109199,
#109200,#109201,#109202,#109203,#109204,#109205,#109206,#109207,#109208,
#109209,#109210,#109211,#109212,#109213,#109214,#109215,#109216,#109217,
#109218,#109219,#109220,#109221,#109222,#109223,#109224,#109225,#109226,
#109227,#109228,#109229,#109230,#109231,#109232,#109233,#109234,#109235,
#109236,#109237,#109238,#109239,#109240,#109241,#109242,#109243,#109244,
#109245,#109246,#109247,#109248,#109249,#109250,#109251,#109252,#109253,
#109254,#109255,#109256,#109257,#109258,#109259,#109260,#109261,#109262,
#109263,#109264,#109265,#109266,#109267,#109268,#109269,#109270,#109271,
#109272,#109273,#109274,#109275,#109276,#109277,#109278,#109279,#109280,
#109281,#109282,#109283,#109284,#109285,#109286,#109287,#109288,#109289,
#109290,#109291,#109292,#109293,#109294,#109295,#109296,#109297,#109298,
#109299,#109300,#109301,#109302,#109303,#109304,#109305,#109306,#109307,
#109308,#109309,#109310,#109311,#109312,#109313,#109314,#109315,#109316,
#109317,#109318,#109319,#109320,#109321,#109322,#109323,#109324,#109325,
#109326,#109327,#109328,#109329,#109330,#109331,#109332,#109333,#109334,
#109335,#109336,#109337,#109338,#109339,#109340,#109341,#109342,#109343,
#109344,#109345,#109346,#109347,#109348,#109349,#109350,#109351,#109352,
#109353,#109354,#109355,#109356,#109357,#109358,#109359,#109360,#109361,
#109362,#109363,#109364,#109365,#109366,#109367,#109368,#109369,#109370,
#109371,#109372,#109373,#109374,#109375,#109376,#109377,#109378,#109379,
#109380,#109381,#109382,#109383,#109384,#109385,#109386,#109387,#109388,
#109389),.UNSPECIFIED.,.F.,.F.,(4,2,2,2,2,2,2,2,2,2,2,2,2,2,2,2,2,2,2,2,
2,2,2,2,2,2,2,2,2,2,2,2,2,2,2,2,2,2,2,2,2,2,2,2,2,2,2,2,2,2,2,2,2,2,2,2,
2,2,2,2,2,2,2,2,2,2,2,2,2,2,2,2,2,2,2,2,2,2,2,2,2,2,2,2,2,2,2,2,2,2,2,2,
2,2,2,2,2,2,2,2,2,2,2,2,2,2,2,2,2,2,4),(-1.40846183573222,-1.36760935404396,
-1.35571677711112,-1.35118168056498,-1.34787326581396,-1.34641078032389,
-1.34532607541812,-1.34413718509467,-1.34217123533643,-1.3357661173238,
-1.33421020789535,-1.31962364758894,-1.26058204198727,-1.2462723306543,
-1.24251063948406,-1.24030180412614,-1.23838914703816,-1.23604641789166,
-1.23155948648072,-1.19919773828322,-1.15901433858493,-1.15408223932826,
-1.13813289937514,-1.13551637136099,-1.13416965978534,-1.13309829372798,
-1.13184088067692,-1.12956413170179,-1.11818557546823,-1.09199672936701,
-1.03927343228281,-1.03235893398958,-1.02948889894336,-1.02769525263767,
-1.02573416548043,-1.02302947935368,-1.01662029543279,-0.988122866940365,
-0.937198879267705,-0.925708217044988,-0.923535237783938,-0.922170811223976,
-0.921098151255365,-0.919853862467044,-0.917637262802063,-0.907255704932003,
-0.884789000923542,-0.826431098724289,-0.820077957807639,-0.817582871117166,
-0.815768411894293,-0.813822913967139,-0.811207586020978,-0.805311225420001,
-0.780924288888288,-0.730257961845517,-0.714076099833773,-0.711449426175511,
-0.710100583030828,-0.709029143525843,-0.707773522827226,-0.705504786963308,
-0.694263711462023,-0.668612691125667,-0.615121987936699,-0.608267484558596,
-0.605407434595423,-0.603615686178932,-0.601653177388932,-0.598940109306859,
-0.592480579174513,-0.538568124541575,-0.502338026817227,-0.499484232452788,
-0.498107390003983,-0.497033673778689,-0.4957980052161,-0.493620530506494,
-0.48383119987943,-0.434918575917131,-0.399786768537606,-0.395499121893788,
-0.392960120996656,-0.391019833082001,-0.388945698678438,-0.385693144596759,
-0.375348089202393,-0.358710841954113,-0.325789830865112,-0.307668578930956,
-0.290154298854215,-0.287477419144722,-0.286117904090707,-0.285045790411848,
-0.283798336677043,-0.281566718793299,-0.270942331211855,-0.247604880567332,
-0.191930349490594,-0.184492974251068,-0.181535148185156,-0.179725544233453,
-0.177896185303057,-0.175387108746966,-0.17004163193405,-0.162936255911303,
-0.1454735968787,-0.0959607259706829,-0.0781787445690996,-0.0754926276015686,
-0.0747637516645625),.UNSPECIFIED.);
#1057=B_SPLINE_CURVE_WITH_KNOTS('',3,(#109390,#109391,#109392,#109393,#109394,
#109395,#109396,#109397,#109398,#109399,#109400,#109401,#109402,#109403,
#109404,#109405,#109406,#109407,#109408,#109409,#109410,#109411,#109412,
#109413,#109414,#109415,#109416,#109417,#109418,#109419,#109420,#109421,
#109422,#109423,#109424,#109425,#109426,#109427,#109428,#109429,#109430,
#109431,#109432,#109433,#109434,#109435,#109436,#109437,#109438,#109439,
#109440,#109441,#109442,#109443,#109444,#109445,#109446,#109447,#109448,
#109449,#109450,#109451,#109452,#109453,#109454,#109455,#109456,#109457,
#109458,#109459,#109460,#109461,#109462,#109463,#109464,#109465,#109466,
#109467,#109468,#109469,#109470,#109471,#109472,#109473,#109474,#109475,
#109476,#109477,#109478,#109479,#109480,#109481,#109482,#109483,#109484,
#109485,#109486,#109487,#109488,#109489,#109490,#109491,#109492,#109493,
#109494,#109495,#109496,#109497,#109498,#109499,#109500,#109501,#109502,
#109503,#109504,#109505,#109506,#109507,#109508,#109509,#109510,#109511,
#109512,#109513,#109514,#109515,#109516,#109517,#109518,#109519,#109520,
#109521,#109522,#109523,#109524,#109525,#109526,#109527,#109528,#109529,
#109530,#109531,#109532,#109533,#109534,#109535,#109536,#109537,#109538,
#109539,#109540,#109541,#109542,#109543,#109544,#109545,#109546,#109547,
#109548,#109549,#109550,#109551,#109552,#109553,#109554,#109555,#109556,
#109557,#109558,#109559,#109560,#109561,#109562,#109563,#109564,#109565,
#109566,#109567,#109568,#109569,#109570,#109571,#109572,#109573,#109574,
#109575,#109576,#109577,#109578,#109579,#109580,#109581,#109582,#109583,
#109584,#109585,#109586,#109587,#109588,#109589,#109590,#109591,#109592,
#109593,#109594,#109595,#109596,#109597,#109598,#109599,#109600,#109601,
#109602,#109603,#109604,#109605,#109606,#109607,#109608,#109609,#109610,
#109611,#109612,#109613,#109614,#109615,#109616,#109617,#109618,#109619,
#109620,#109621,#109622,#109623,#109624,#109625,#109626,#109627,#109628,
#109629,#109630,#109631,#109632,#109633,#109634,#109635,#109636,#109637,
#109638,#109639,#109640,#109641,#109642,#109643,#109644,#109645,#109646,
#109647,#109648,#109649,#109650,#109651,#109652,#109653,#109654,#109655,
#109656,#109657,#109658,#109659),.UNSPECIFIED.,.F.,.F.,(4,2,2,2,2,2,2,2,
2,2,2,2,2,2,2,2,2,2,2,2,2,2,2,2,2,2,2,2,2,2,2,2,2,2,2,2,2,2,2,2,2,2,2,2,
2,2,2,2,2,2,2,2,2,2,2,2,2,2,2,2,2,2,2,2,2,2,2,2,2,2,2,2,2,2,2,2,2,2,2,2,
2,2,2,2,2,2,2,2,2,2,2,2,2,2,2,2,2,2,2,2,2,2,2,2,2,2,2,2,2,2,2,2,2,2,2,2,
2,2,2,2,2,2,2,2,2,2,2,2,2,2,2,2,2,2,4),(-2.59345435029626,-2.57487343302133,
-2.55603054349818,-2.54673538719394,-2.54459246186581,-2.54336430675748,
-2.54228927408724,-2.54090039316212,-2.53798547053879,-2.50828829265839,
-2.45783806134818,-2.448348849042,-2.44374148092713,-2.43996230701688,-2.43779156057653,
-2.43777586588201,-2.4377596186006,-2.43774279865574,-2.43772538517487,
-2.43770735653761,-2.4376886903526,-2.43766936342921,-2.43764935173658,
-2.43762863030754,-2.43760717336548,-2.43758495418478,-2.43756194437979,
-2.4375419078355,-2.43751855724927,-2.43749135053028,-2.43745965963862,
-2.43742275825009,-2.43737980810024,-2.43732559577303,-2.43538484296361,
-2.4328427911657,-2.42854454965186,-2.39342281925613,-2.34446396997995,
-2.33476354132117,-2.33259226802617,-2.33135800420501,-2.33028415775527,
-2.32890537102029,-2.32604143566114,-2.29008480882023,-2.25731885641484,
-2.23475907357195,-2.2291055815852,-2.22653436290148,-2.22459595571837,
-2.22276929615355,-2.22022742796077,-2.21358646657787,-2.15778055934402,
-2.13371804059057,-2.12289465798696,-2.12065069774379,-2.11940046807973,
-2.1183285190827,-2.1169724785515,-2.11482692102098,-2.103790203029,-2.05257229344681,
-2.02386280264726,-2.01742903107829,-2.01472032560763,-2.01275863406502,
-2.01096602804043,-2.0081011128712,-2.0012168098453,-1.94814075254518,-1.92223332524728,
-1.91092603288176,-1.9086535387874,-1.90739711624071,-1.90632577261868,
-1.9049780372029,-1.9023564291846,-1.88631425680576,-1.88102344571043,-1.86643879725074,
-1.83354645597647,-1.81697937446422,-1.80666682974584,-1.8034178286264,
-1.80134436492348,-1.79940358499364,-1.79686232702021,-1.79256728680515,
-1.75745480157287,-1.70854954716936,-1.69877886429716,-1.69660261330852,
-1.69536717676263,-1.6942933711541,-1.69291602419614,-1.69005985817146,
-1.6672595939259,-1.61165016670609,-1.59563848503265,-1.59186896715905,
-1.58968046471779,-1.58776623391067,-1.58539691891518,-1.5817634981857,
-1.564666135491,-1.5565973928003,-1.52178644924782,-1.49773633287172,-1.48691654931937,
-1.48467289985831,-1.48342278231305,-1.48235089181459,-1.48099487700528,
-1.47833455998944,-1.46128086936533,-1.44266851361881,-1.4097118208564,
-1.39306633846209,-1.38271848467888,-1.37946551532565,-1.37739123382153,
-1.3754508914063,-1.37291194014815,-1.3686246799394,-1.33404296401158,-1.27807638839781,
-1.27380249806267,-1.27213089678816,-1.27111885272133,-1.27001650027444,
-1.26845155766493,-1.26453897460501,-1.25988555695749),.UNSPECIFIED.);
#1058=B_SPLINE_CURVE_WITH_KNOTS('',3,(#109665,#109666,#109667,#109668,#109669,
#109670,#109671,#109672,#109673,#109674,#109675,#109676,#109677,#109678,
#109679,#109680,#109681,#109682),.UNSPECIFIED.,.F.,.F.,(4,2,2,2,2,2,2,2,
4),(-0.0751187269598587,-0.0651105008529126,-0.0603738607500047,-0.057948073480137,
-0.0560290632015776,-0.0538783934967688,-0.0516516909504345,-0.0483298717746776,
-0.000628983924256894),.UNSPECIFIED.);
#1059=B_SPLINE_CURVE_WITH_KNOTS('',3,(#109683,#109684,#109685,#109686,#109687,
#109688,#109689,#109690,#109691,#109692,#109693,#109694,#109695,#109696,
#109697,#109698,#109699,#109700,#109701,#109702,#109703,#109704,#109705,
#109706,#109707,#109708,#109709,#109710,#109711,#109712,#109713,#109714,
#109715,#109716,#109717,#109718,#109719,#109720,#109721,#109722,#109723,
#109724,#109725,#109726,#109727,#109728,#109729,#109730,#109731,#109732,
#109733,#109734,#109735,#109736,#109737,#109738,#109739,#109740,#109741,
#109742,#109743,#109744,#109745,#109746,#109747,#109748,#109749,#109750,
#109751,#109752,#109753,#109754,#109755,#109756,#109757,#109758,#109759,
#109760,#109761,#109762,#109763,#109764,#109765,#109766,#109767,#109768,
#109769,#109770,#109771,#109772,#109773,#109774,#109775,#109776,#109777,
#109778,#109779,#109780,#109781,#109782,#109783,#109784,#109785,#109786,
#109787,#109788,#109789,#109790,#109791,#109792,#109793,#109794,#109795,
#109796,#109797,#109798,#109799,#109800,#109801,#109802,#109803,#109804,
#109805,#109806,#109807,#109808,#109809,#109810,#109811,#109812,#109813,
#109814,#109815,#109816,#109817,#109818,#109819,#109820,#109821,#109822,
#109823,#109824,#109825,#109826,#109827,#109828,#109829,#109830,#109831,
#109832,#109833,#109834,#109835,#109836,#109837,#109838,#109839,#109840,
#109841,#109842,#109843,#109844,#109845,#109846,#109847,#109848,#109849,
#109850,#109851,#109852,#109853,#109854,#109855,#109856,#109857,#109858,
#109859,#109860,#109861,#109862,#109863,#109864,#109865,#109866,#109867,
#109868,#109869,#109870,#109871,#109872,#109873,#109874,#109875,#109876,
#109877,#109878,#109879,#109880,#109881,#109882,#109883,#109884,#109885,
#109886,#109887,#109888,#109889,#109890,#109891,#109892,#109893,#109894,
#109895,#109896,#109897,#109898,#109899,#109900,#109901,#109902,#109903,
#109904,#109905,#109906,#109907,#109908,#109909,#109910),.UNSPECIFIED.,
 .F.,.F.,(4,2,2,2,2,2,2,2,2,2,2,2,2,2,2,2,2,2,2,2,2,2,2,2,2,2,2,2,2,2,2,
2,2,2,2,2,2,2,2,2,2,2,2,2,2,2,2,2,2,2,2,2,2,2,2,2,2,2,2,2,2,2,2,2,2,2,2,
2,2,2,2,2,2,2,2,2,2,2,2,2,2,2,2,2,2,2,2,2,2,2,2,2,2,2,2,2,2,2,2,2,2,2,2,
2,2,2,2,2,2,2,2,2,2,4),(-2.66766695993853,-2.62471357151963,-2.62177987548942,
-2.62009725320902,-2.61859242480639,-2.61750086530987,-2.61647356640042,
-2.61472395506007,-2.60994937627041,-2.57250172672594,-2.55111738233075,
-2.52297782877626,-2.51633382567163,-2.51419350871687,-2.51210259779417,
-2.51016781385845,-2.50766602902802,-2.50350712852976,-2.47508598865391,
-2.44452441819042,-2.42045245241616,-2.40964062699257,-2.40740758394692,
-2.4061496438327,-2.40507822136512,-2.40373193197073,-2.40111767193013,
-2.38522589855565,-2.38061496893986,-2.332214992904,-2.3156705597439,-2.30540677793349,
-2.30223450532698,-2.30013654154442,-2.29820421266851,-2.29571814072694,
-2.29161244469763,-2.26523392152814,-2.21006137226532,-2.19772551770827,
-2.1953966964881,-2.19412793620628,-2.19305724478535,-2.19172438264602,
-2.18965484953988,-2.17978309477761,-2.17405469228903,-2.16659958338089,
-2.16525949738652,-2.12103637417534,-2.09759236277211,-2.09181977710513,
-2.08922645996908,-2.08728424122182,-2.08546334837626,-2.08294440099943,
-2.07644869911415,-2.01926568033057,-2.01353564816784,-1.99465320548339,
-1.98534514768651,-1.98320113692008,-1.98197266386553,-1.98089755124883,
-1.97950882881032,-1.97659516278302,-1.94769410723579,-1.91155771415965,
-1.89277977092843,-1.88149522970752,-1.87813877271382,-1.87604132388002,
-1.87410852573285,-1.8716205354189,-1.86750883815242,-1.84091458245761,
-1.79877356684269,-1.78189820759751,-1.77324820062156,-1.77115367064405,
-1.76993613341275,-1.7688589834256,-1.76747550605699,-1.76519026255414,
-1.75159291516044,-1.74979364095306,-1.70242181693978,-1.6714466509955,
-1.66699463761633,-1.66465901159815,-1.66274651804397,-1.66053154277795,
-1.65674398699093,-1.64214946712625,-1.62988390412784,-1.58947273110877,
-1.5706189598816,-1.56132013229282,-1.5591768459171,-1.55794856209121,-1.55687346777172,
-1.55548457454187,-1.55256986386833,-1.52373234564028,-1.48562133855473,
-1.46809570978883,-1.4573545763476,-1.45405689616496,-1.45197248113065,
-1.45003539428428,-1.44751885764649,-1.44330959396303,-1.41283498024576,
-1.40846183573222),.UNSPECIFIED.);
#1060=B_SPLINE_CURVE_WITH_KNOTS('',3,(#109912,#109913,#109914,#109915,#109916,
#109917,#109918,#109919,#109920,#109921,#109922,#109923,#109924,#109925,
#109926,#109927,#109928,#109929,#109930,#109931,#109932,#109933,#109934,
#109935,#109936,#109937,#109938,#109939,#109940,#109941,#109942,#109943,
#109944,#109945,#109946,#109947,#109948,#109949,#109950,#109951,#109952,
#109953,#109954,#109955,#109956,#109957,#109958,#109959,#109960,#109961,
#109962,#109963,#109964,#109965,#109966,#109967,#109968,#109969,#109970,
#109971,#109972,#109973,#109974,#109975,#109976,#109977,#109978,#109979,
#109980,#109981,#109982,#109983,#109984,#109985,#109986,#109987,#109988,
#109989,#109990,#109991,#109992,#109993,#109994,#109995,#109996,#109997,
#109998,#109999,#110000,#110001,#110002,#110003,#110004,#110005,#110006,
#110007,#110008,#110009,#110010,#110011,#110012,#110013,#110014,#110015,
#110016,#110017,#110018,#110019,#110020,#110021,#110022,#110023,#110024,
#110025,#110026,#110027,#110028,#110029,#110030,#110031,#110032,#110033,
#110034,#110035,#110036,#110037,#110038,#110039,#110040,#110041,#110042,
#110043,#110044,#110045,#110046,#110047,#110048,#110049,#110050,#110051,
#110052,#110053,#110054,#110055,#110056,#110057,#110058,#110059,#110060,
#110061,#110062,#110063,#110064,#110065,#110066,#110067,#110068,#110069,
#110070,#110071,#110072,#110073,#110074,#110075,#110076,#110077,#110078,
#110079,#110080,#110081,#110082,#110083,#110084,#110085,#110086,#110087,
#110088,#110089,#110090,#110091,#110092,#110093,#110094,#110095,#110096,
#110097,#110098,#110099,#110100,#110101,#110102,#110103,#110104,#110105,
#110106,#110107,#110108,#110109,#110110,#110111,#110112,#110113,#110114,
#110115,#110116,#110117,#110118,#110119,#110120,#110121,#110122,#110123,
#110124,#110125,#110126,#110127,#110128,#110129,#110130,#110131,#110132,
#110133,#110134,#110135,#110136,#110137,#110138,#110139,#110140,#110141,
#110142,#110143,#110144,#110145,#110146,#110147,#110148,#110149,#110150,
#110151,#110152,#110153,#110154,#110155,#110156,#110157,#110158,#110159,
#110160,#110161,#110162,#110163,#110164,#110165,#110166,#110167),
 .UNSPECIFIED.,.F.,.F.,(4,2,2,2,2,2,2,2,2,2,2,2,2,2,2,2,2,2,2,2,2,2,2,2,
2,2,2,2,2,2,2,2,2,2,2,2,2,2,2,2,2,2,2,2,2,2,2,2,2,2,2,2,2,2,2,2,2,2,2,2,
2,2,2,2,2,2,2,2,2,2,2,2,2,2,2,2,2,2,2,2,2,2,2,2,2,2,2,2,2,2,2,2,2,2,2,2,
2,2,2,2,2,2,2,2,2,2,2,2,2,2,2,2,2,2,2,2,2,2,2,2,2,2,2,2,2,2,2,4),(-1.25988555695749,
-1.24532638527379,-1.18895160322942,-1.17210635115282,-1.16848959436862,
-1.16612546470395,-1.16421164300566,-1.1620194592878,-1.15823310554555,
-1.14198618534886,-1.08451057375482,-1.07953846025835,-1.06355310283422,
-1.06093472943854,-1.0595876590446,-1.05851631858572,-1.05725929627782,
-1.05498417256997,-1.04363264697203,-1.01754955677824,-0.964679565391793,
-0.957776503627436,-0.954908435567873,-0.953115209880324,-0.951153933219339,
-0.948447796236104,-0.942029554150818,-0.913455071828924,-0.862260476417587,
-0.851097438988294,-0.848944131514223,-0.847585723903216,-0.846513593116859,
-0.845265097591007,-0.843029080127315,-0.832336174459459,-0.808751048046474,
-0.752171282267619,-0.745607594149311,-0.743077980625541,-0.741254558118842,
-0.739314439323958,-0.736732147990228,-0.73101815388237,-0.708011594626844,
-0.674988410250267,-0.653838201291532,-0.6394335828407,-0.637109688979565,
-0.635715078715253,-0.634636814177033,-0.633426476253124,-0.631363222198257,
-0.623097286303419,-0.607329663075481,-0.565247540525825,-0.537107798038922,
-0.532957134485539,-0.53045815685201,-0.528524264249283,-0.526433043031681,
-0.523102592125976,-0.512054873399786,-0.493827900162138,-0.444883046408736,
-0.427669885066384,-0.425003850105975,-0.423646647400107,-0.422574708937565,
-0.421325565883563,-0.419086221032513,-0.408336392100513,-0.384541072611784,
-0.328294934455361,-0.32169691908426,-0.319161979739908,-0.317337273738358,
-0.315398148959251,-0.312821212149841,-0.307135635914288,-0.284338654622944,
-0.233331782369013,-0.231142533946231,-0.215562932255187,-0.212983041122076,
-0.211659059758323,-0.210638858375426,-0.210630841871536,-0.21062299470742,
-0.210615306447954,-0.210607767556776,-0.210600369080208,-0.21059310271116,
-0.210585960810013,-0.210578936212478,-0.210572022261058,-0.210565212726491,
-0.210558501849934,-0.210551884105566,-0.210545354392377,-0.21053890772416,
-0.210532539685671,-0.210526245983347,-0.210520022512278,-0.210513865397359,
-0.21050777101508,-0.210501735916263,-0.210495756758664,-0.21048983061208,
-0.210483954282331,-0.210478124871857,-0.209215188219218,-0.206828581169588,
-0.193289889053911,-0.157226498309435,-0.113379973391436,-0.109095331437991,
-0.106557349953289,-0.104617402728217,-0.102543206822558,-0.099289665684863,
-0.0889339236456346,-0.0722722792900259,-0.041786616349719,-0.00539386482498733,
-0.00193475652062522,-0.000864055931841007,-0.000629064156325977),
 .UNSPECIFIED.);
#1061=B_SPLINE_CURVE_WITH_KNOTS('',3,(#110168,#110169,#110170,#110171,#110172,
#110173,#110174,#110175,#110176,#110177,#110178,#110179,#110180,#110181,
#110182,#110183),.UNSPECIFIED.,.F.,.F.,(4,3,3,3,3,4),(-28.973780262141,
-28.9662570488944,-28.8628842312382,-28.7596459043713,-28.6565264336345,
-28.6232428877577),.UNSPECIFIED.);
#1062=B_SPLINE_CURVE_WITH_KNOTS('',3,(#110188,#110189,#110190,#110191,#110192,
#110193,#110194,#110195,#110196,#110197,#110198,#110199,#110200,#110201,
#110202,#110203,#110204,#110205,#110206,#110207,#110208,#110209,#110210,
#110211,#110212,#110213,#110214,#110215,#110216,#110217,#110218,#110219,
#110220,#110221,#110222,#110223,#110224,#110225,#110226,#110227,#110228,
#110229,#110230,#110231,#110232,#110233,#110234,#110235,#110236,#110237,
#110238,#110239,#110240,#110241,#110242,#110243,#110244,#110245,#110246,
#110247,#110248,#110249,#110250,#110251,#110252,#110253,#110254,#110255,
#110256,#110257,#110258,#110259,#110260,#110261,#110262,#110263,#110264,
#110265,#110266,#110267,#110268,#110269,#110270,#110271,#110272,#110273,
#110274,#110275,#110276,#110277,#110278,#110279,#110280,#110281,#110282,
#110283,#110284,#110285,#110286,#110287,#110288,#110289,#110290,#110291,
#110292,#110293,#110294,#110295,#110296,#110297,#110298,#110299,#110300,
#110301,#110302,#110303,#110304,#110305,#110306,#110307,#110308,#110309,
#110310,#110311,#110312,#110313,#110314,#110315,#110316,#110317,#110318,
#110319,#110320,#110321,#110322,#110323,#110324,#110325,#110326,#110327,
#110328,#110329,#110330,#110331,#110332,#110333,#110334,#110335,#110336,
#110337,#110338,#110339,#110340,#110341,#110342,#110343,#110344,#110345,
#110346,#110347,#110348,#110349,#110350,#110351,#110352,#110353,#110354,
#110355,#110356,#110357,#110358,#110359,#110360,#110361,#110362,#110363,
#110364,#110365,#110366,#110367,#110368,#110369,#110370,#110371,#110372,
#110373,#110374,#110375,#110376,#110377,#110378,#110379,#110380,#110381,
#110382,#110383,#110384,#110385,#110386,#110387,#110388,#110389,#110390,
#110391,#110392,#110393,#110394,#110395,#110396,#110397,#110398,#110399,
#110400,#110401,#110402,#110403,#110404,#110405,#110406,#110407,#110408,
#110409,#110410,#110411,#110412,#110413,#110414,#110415,#110416,#110417),
 .UNSPECIFIED.,.F.,.F.,(4,2,2,2,2,2,2,2,2,2,2,2,2,2,2,2,2,2,2,2,2,2,2,2,
2,2,2,2,2,2,2,2,2,2,2,2,2,2,2,2,2,2,2,2,2,2,2,2,2,2,2,2,2,2,2,2,2,2,2,2,
2,2,2,2,2,2,2,2,2,2,2,2,2,2,2,2,2,2,2,2,2,2,2,2,2,2,2,2,2,2,2,2,2,2,2,2,
2,2,2,2,2,2,2,2,2,2,2,2,2,2,2,2,2,2,4),(-1.40849963608456,-1.36250086534813,
-1.34494541177015,-1.33419124570262,-1.33089220484147,-1.32880754118493,
-1.32687064546567,-1.32431146871617,-1.31872496522311,-1.31130161884544,
-1.29270004945226,-1.24997196002806,-1.22734421722922,-1.22449209291687,
-1.22311545919613,-1.22204162478914,-1.22080550277749,-1.21862646861658,
-1.20881749322397,-1.15991304437755,-1.12479441280277,-1.12049879708814,
-1.11795729616835,-1.11601637595224,-1.1139428053469,-1.11069372524074,
-1.10038159156822,-1.08381810755195,-1.05095542944343,-1.03712730217916,
-1.0304779110454,-1.015004310628,-1.01240725994416,-1.01106477504636,-1.009993699204,
-1.00873305094366,-1.00644128609784,-0.994794933060641,-0.967529635336812,
-0.94734520946427,-0.91283762636,-0.908551009330935,-0.906012141320413,
-0.904071679935995,-0.901997093043025,-0.898743270755462,-0.888389449269371,
-0.871733584457522,-0.83879471098802,-0.820070761551213,-0.803158031315011,
-0.800502885531302,-0.799147913410304,-0.798076020379622,-0.796824954757866,
-0.794577229742132,-0.783692553638892,-0.759399756619677,-0.703899136882833,
-0.697223955902817,-0.6946767164775,-0.692848614562407,-0.690910896837158,
-0.688344354483421,-0.682716407593117,-0.675222993875717,-0.656363960129019,
-0.626392479024081,-0.604467361698181,-0.590931231729453,-0.58864953436849,
-0.587267326295838,-0.586190619468233,-0.584972979309737,-0.582876886936892,
-0.574201278309242,-0.55724515214131,-0.515316336921049,-0.488613915676676,
-0.484500237825154,-0.482012098258073,-0.480079798313352,-0.477983504499995,
-0.47463023154339,-0.463368913111905,-0.444645514487062,-0.416442756046856,
-0.379487469877617,-0.376649028657838,-0.375275309310357,-0.374202004849005,
-0.372964519233759,-0.370778337042213,-0.361231512847888,-0.312154875908352,
-0.276986654722135,-0.272691439467162,-0.270150410452519,-0.268209985932634,
-0.266137076081078,-0.262889305186038,-0.252778852228058,-0.236574643820261,
-0.198328907679375,-0.167652335660903,-0.164739947093335,-0.163351838761409,
-0.162277200155732,-0.161049276403844,-0.159757267870224,-0.155110071595339,
-0.128864883766184,-0.10699088015377,-0.105559722238614,-0.0751187269598587),
 .UNSPECIFIED.);
#1063=B_SPLINE_CURVE_WITH_KNOTS('',3,(#110419,#110420,#110421,#110422,#110423,
#110424,#110425,#110426,#110427,#110428,#110429,#110430,#110431,#110432,
#110433,#110434,#110435,#110436,#110437,#110438,#110439,#110440,#110441,
#110442,#110443,#110444,#110445,#110446,#110447,#110448,#110449,#110450,
#110451,#110452,#110453,#110454,#110455,#110456,#110457,#110458,#110459,
#110460,#110461,#110462,#110463,#110464,#110465,#110466,#110467,#110468,
#110469,#110470,#110471,#110472,#110473,#110474,#110475,#110476,#110477,
#110478,#110479,#110480,#110481,#110482,#110483,#110484,#110485,#110486,
#110487,#110488,#110489,#110490,#110491,#110492,#110493,#110494,#110495,
#110496,#110497,#110498,#110499,#110500,#110501,#110502,#110503,#110504,
#110505,#110506,#110507,#110508,#110509,#110510,#110511,#110512,#110513,
#110514,#110515,#110516,#110517,#110518,#110519,#110520,#110521,#110522,
#110523,#110524,#110525,#110526,#110527,#110528,#110529,#110530,#110531,
#110532,#110533,#110534,#110535,#110536,#110537,#110538,#110539,#110540,
#110541,#110542,#110543,#110544,#110545,#110546,#110547,#110548,#110549,
#110550,#110551,#110552,#110553,#110554,#110555,#110556,#110557,#110558,
#110559,#110560,#110561,#110562,#110563,#110564,#110565,#110566,#110567,
#110568,#110569,#110570,#110571,#110572,#110573,#110574,#110575,#110576,
#110577,#110578,#110579,#110580,#110581,#110582,#110583,#110584,#110585,
#110586,#110587,#110588,#110589,#110590,#110591,#110592,#110593,#110594,
#110595,#110596,#110597,#110598,#110599),.UNSPECIFIED.,.F.,.F.,(4,3,3,3,
3,3,3,3,3,3,3,3,3,3,3,3,3,3,3,3,3,3,3,3,3,3,3,3,3,3,3,3,3,3,3,3,3,3,3,3,
3,3,3,3,3,3,3,3,3,3,3,3,3,3,3,3,3,3,3,3,4),(-28.6232428877577,-28.5202021552005,
-28.4171818104866,-28.3141478661896,-28.2110002753443,-28.1077865067903,
-28.0043999094814,-27.9674205989325,-27.8640258618989,-27.7607845797986,
-27.6576646144211,-27.554610046227,-27.4515868378843,-27.3485609952268,
-27.2454282284638,-27.142239137069,-27.0388671437024,-26.9685841489706,
-26.8651894118469,-26.761948129656,-26.6588281641879,-26.5557735959032,
-26.4527503874699,-26.3497245447222,-26.2465917778698,-26.1434026863862,
-26.0400306929323,-25.9697476990087,-25.8663529620654,-25.7631116800547,
-25.6599917147658,-25.5569371466596,-25.4539139384038,-25.3508880958323,
-25.2477553291532,-25.1445662378413,-25.0411942445548,-24.9709112490468,
-24.8675165120618,-24.7642752300111,-24.6611552646847,-24.5581006965428,
-24.4550774882529,-24.352051645649,-24.2489188789403,-24.1457297876004,
-24.0423577942887,-23.972074799085,-23.8686800615172,-23.7654387788806,
-23.6623188129668,-23.5592642442367,-23.4562410353589,-23.353215192168,
-23.2500824248778,-23.1468933329587,-23.0435213390778,-22.9732383491231,
-22.8444301460683,-22.7177283292801,-22.6905949549614),.UNSPECIFIED.);
#1064=B_SPLINE_CURVE_WITH_KNOTS('',3,(#110600,#110601,#110602,#110603),
 .UNSPECIFIED.,.F.,.F.,(4,4),(-22.6905949549614,-22.3411473650526),
 .UNSPECIFIED.);
#1065=B_SPLINE_CURVE_WITH_KNOTS('',3,(#110609,#110610,#110611,#110612,#110613,
#110614,#110615,#110616,#110617,#110618,#110619,#110620,#110621,#110622,
#110623,#110624,#110625,#110626),.UNSPECIFIED.,.F.,.F.,(4,2,2,2,2,2,2,2,
4),(-0.0747374496497559,-0.0441237844182805,-0.0412117011286783,-0.0398236116774997,
-0.0387489292896549,-0.0375208900578933,-0.0362287396242862,-0.0342507365147655,
-0.000628701287238877),.UNSPECIFIED.);
#1066=B_SPLINE_CURVE_WITH_KNOTS('',3,(#110627,#110628,#110629,#110630,#110631,
#110632,#110633,#110634,#110635,#110636,#110637,#110638,#110639,#110640,
#110641,#110642,#110643,#110644,#110645,#110646,#110647,#110648,#110649,
#110650,#110651,#110652,#110653,#110654,#110655,#110656,#110657,#110658,
#110659,#110660,#110661,#110662,#110663,#110664,#110665,#110666,#110667,
#110668,#110669,#110670,#110671,#110672,#110673,#110674,#110675,#110676,
#110677,#110678,#110679,#110680,#110681,#110682,#110683,#110684,#110685,
#110686,#110687,#110688,#110689,#110690,#110691,#110692,#110693,#110694,
#110695,#110696,#110697,#110698,#110699,#110700,#110701,#110702,#110703,
#110704,#110705,#110706,#110707,#110708,#110709,#110710,#110711,#110712,
#110713,#110714,#110715,#110716,#110717,#110718,#110719,#110720,#110721,
#110722,#110723,#110724,#110725,#110726,#110727,#110728,#110729,#110730,
#110731,#110732,#110733,#110734,#110735,#110736,#110737,#110738,#110739,
#110740,#110741,#110742,#110743,#110744,#110745,#110746,#110747,#110748,
#110749,#110750,#110751,#110752,#110753,#110754,#110755,#110756,#110757,
#110758,#110759,#110760,#110761,#110762,#110763,#110764,#110765,#110766,
#110767,#110768,#110769,#110770,#110771,#110772,#110773,#110774,#110775,
#110776,#110777,#110778,#110779,#110780,#110781,#110782,#110783,#110784,
#110785,#110786,#110787,#110788,#110789,#110790,#110791,#110792,#110793,
#110794,#110795,#110796,#110797,#110798,#110799,#110800,#110801,#110802,
#110803,#110804,#110805,#110806,#110807,#110808,#110809,#110810,#110811,
#110812,#110813,#110814,#110815,#110816,#110817,#110818,#110819,#110820,
#110821,#110822,#110823,#110824,#110825,#110826,#110827,#110828,#110829,
#110830,#110831,#110832,#110833,#110834,#110835,#110836,#110837,#110838,
#110839,#110840,#110841,#110842,#110843,#110844,#110845,#110846),
 .UNSPECIFIED.,.F.,.F.,(4,2,2,2,2,2,2,2,2,2,2,2,2,2,2,2,2,2,2,2,2,2,2,2,
2,2,2,2,2,2,2,2,2,2,2,2,2,2,2,2,2,2,2,2,2,2,2,2,2,2,2,2,2,2,2,2,2,2,2,2,
2,2,2,2,2,2,2,2,2,2,2,2,2,2,2,2,2,2,2,2,2,2,2,2,2,2,2,2,2,2,2,2,2,2,2,2,
2,2,2,2,2,2,2,2,2,2,2,2,2,4),(-2.66802542164946,-2.63755417114925,-2.61103832252004,
-2.60487114890265,-2.60220785653925,-2.60025403454764,-2.59845111805707,
-2.59553095236573,-2.58831615461444,-2.54291362715924,-2.52278252471317,
-2.50656823983998,-2.49817190163438,-2.49612451106828,-2.49489637664954,
-2.4938213787511,-2.4924325646186,-2.48951785900045,-2.45949080718715,-2.4082036857542,
-2.39936634425664,-2.3929590848947,-2.39025468606481,-2.38829361857624,
-2.38649986413826,-2.38362936940678,-2.37671225829577,-2.32405732039061,
-2.29784926700888,-2.28646513786489,-2.28418807232359,-2.2829305762518,
-2.28185919856569,-2.28051254141557,-2.27789632360918,-2.26195362471783,
-2.25752409833991,-2.21497018184428,-2.18434635016617,-2.17990434965435,
-2.1775709988326,-2.17565885536641,-2.17344258182554,-2.1696486409106,-2.15497835789923,
-2.14272676364302,-2.10721191288641,-2.0847663655952,-2.07439005645545,
-2.07217382100489,-2.0709296132986,-2.0698569503543,-2.06849241762192,-2.06579252371313,
-2.04761342823916,-2.02952741803248,-1.99679663800888,-1.97429543162791,
-1.96864952379694,-1.96607949520937,-1.9641410649718,-1.96231370703854,
-1.95976978044937,-1.95311694568588,-1.89740855395777,-1.87327422033005,
-1.86243090428267,-1.86018552488489,-1.85893488430517,-1.85786281704301,
-1.85650692708351,-1.85436217006904,-1.84334150555545,-1.79204137555043,
-1.76337564037632,-1.7569466818527,-1.75423857360005,-1.75227679575202,
-1.75048375393106,-1.74761736581653,-1.74072550021672,-1.68772904682384,
-1.66175792437525,-1.65043377730957,-1.64816010019916,-1.64690331971634,
-1.64583185063414,-1.64448418622504,-1.64186338936202,-1.62583795685175,
-1.62043989082364,-1.60593640459328,-1.573040655047,-1.55028407741119,-1.54460348675651,
-1.54202698421215,-1.54008744859317,-1.53826181943444,-1.53572473920949,
-1.52911608717087,-1.47296631352672,-1.44911719837533,-1.43835070904764,
-1.43610988788624,-1.43486018851902,-1.43378794177061,-1.43243055848784,
-1.4297648025452,-1.41257812712104,-1.40849963608456),.UNSPECIFIED.);
#1067=B_SPLINE_CURVE_WITH_KNOTS('',3,(#110848,#110849,#110850,#110851,#110852,
#110853,#110854,#110855,#110856,#110857),.UNSPECIFIED.,.F.,.F.,(4,1,1,1,
1,1,1,4),(-22.3411473650526,-21.9744018991612,-20.9755654491994,-19.9767289992375,
-18.9778925492756,-17.9790560993137,-16.9802196493519,-16.4074096477818),
 .UNSPECIFIED.);
#1068=B_SPLINE_CURVE_WITH_KNOTS('',3,(#110858,#110859,#110860,#110861,#110862,
#110863),.UNSPECIFIED.,.F.,.F.,(4,2,4),(-2.66742166919024,-2.60891629842673,
-2.59315592110003),.UNSPECIFIED.);
#1069=B_SPLINE_CURVE_WITH_KNOTS('',3,(#110868,#110869,#110870,#110871,#110872,
#110873,#110874,#110875,#110876,#110877,#110878,#110879,#110880,#110881,
#110882,#110883,#110884,#110885,#110886,#110887,#110888,#110889,#110890,
#110891,#110892,#110893,#110894,#110895,#110896,#110897,#110898,#110899,
#110900,#110901,#110902,#110903,#110904,#110905,#110906,#110907,#110908,
#110909,#110910,#110911,#110912,#110913,#110914,#110915,#110916,#110917,
#110918,#110919,#110920,#110921,#110922,#110923,#110924,#110925,#110926,
#110927,#110928,#110929,#110930,#110931,#110932,#110933,#110934,#110935,
#110936,#110937,#110938,#110939,#110940,#110941,#110942,#110943,#110944,
#110945,#110946,#110947,#110948,#110949,#110950,#110951,#110952,#110953,
#110954,#110955,#110956,#110957,#110958,#110959,#110960,#110961,#110962,
#110963,#110964,#110965,#110966,#110967,#110968,#110969,#110970,#110971,
#110972,#110973,#110974,#110975,#110976,#110977,#110978,#110979,#110980,
#110981,#110982,#110983,#110984,#110985,#110986,#110987,#110988,#110989,
#110990,#110991,#110992,#110993,#110994,#110995,#110996,#110997,#110998,
#110999,#111000,#111001,#111002,#111003,#111004,#111005,#111006,#111007,
#111008,#111009,#111010,#111011,#111012,#111013,#111014,#111015,#111016,
#111017,#111018,#111019,#111020,#111021,#111022,#111023,#111024,#111025,
#111026,#111027,#111028,#111029,#111030,#111031,#111032,#111033,#111034,
#111035,#111036,#111037,#111038,#111039,#111040,#111041,#111042,#111043,
#111044,#111045,#111046,#111047,#111048,#111049,#111050,#111051,#111052,
#111053,#111054,#111055,#111056,#111057,#111058,#111059,#111060,#111061,
#111062,#111063,#111064,#111065,#111066,#111067,#111068,#111069,#111070,
#111071,#111072,#111073,#111074,#111075,#111076,#111077,#111078,#111079,
#111080,#111081,#111082,#111083,#111084,#111085,#111086,#111087,#111088,
#111089,#111090,#111091),.UNSPECIFIED.,.F.,.F.,(4,2,2,2,2,2,2,2,2,2,2,2,
2,2,2,2,2,2,2,2,2,2,2,2,2,2,2,2,2,2,2,2,2,2,2,2,2,2,2,2,2,2,2,2,2,2,2,2,
2,2,2,2,2,2,2,2,2,2,2,2,2,2,2,2,2,2,2,2,2,2,2,2,2,2,2,2,2,2,2,2,2,2,2,2,
2,2,2,2,2,2,2,2,2,2,2,2,2,2,2,2,2,2,2,2,2,2,2,2,2,2,2,4),(-1.40825517075566,
-1.36486070561898,-1.33380956985227,-1.31575891231249,-1.31306317661106,
-1.31169947357094,-1.31062680438786,-1.30938183875461,-1.30716243548391,
-1.29673882022339,-1.27412454479273,-1.21599821858833,-1.20961431155974,
-1.20711395446872,-1.20529802421571,-1.20335316480793,-1.20074255280682,
-1.19487327385787,-1.17069584189302,-1.12021061713001,-1.11977980004809,
-1.10359243152392,-1.10096535738956,-1.09961635537938,-1.09854481881298,
-1.09728912007681,-1.0950203123576,-1.08378027973149,-1.05813476867367,
-1.00462903004577,-0.997774874658043,-0.994914745537326,-0.993122882415104,
-0.991160195526036,-0.988446784775229,-0.981985979620462,-0.928043982984161,
-0.891838135733603,-0.888983288922922,-0.887606177339344,-0.88653236320879,
-0.885296708443276,-0.883119562402402,-0.873336757335368,-0.824414215182172,
-0.789290664026276,-0.784995243414214,-0.782453888004092,-0.780513096273503,
-0.778439679793219,-0.775190876441804,-0.764879919409157,-0.748318611586668,
-0.715459017225508,-0.701719286163376,-0.694865970527898,-0.694544051345743,
-0.68882747734314,-0.678952475356014,-0.676883015550683,-0.675550313355996,
-0.674479832973003,-0.673211423550649,-0.670883507061314,-0.65855923581904,
-0.603512539575028,-0.576984973962758,-0.572875855777599,-0.570389091677128,
-0.568457036580506,-0.566360183106348,-0.563004217864846,-0.551716844864075,
-0.532932223090572,-0.497974924995506,-0.467987713472837,-0.465074023301411,
-0.463685608444667,-0.462610877514032,-0.461383010982414,-0.459240440159017,
-0.449944824800894,-0.431095093403466,-0.387250853073146,-0.364754422847273,
-0.360810609394575,-0.358346530092496,-0.356423149017978,-0.354294224281466,
-0.350793180911979,-0.338041041544176,-0.315661048082141,-0.265630907114065,
-0.255111362957835,-0.252998938797095,-0.251653126764957,-0.250582034471614,
-0.24932442991037,-0.247091844486272,-0.236304903717156,-0.212308631438729,
-0.186250529351654,-0.153387327652072,-0.149130333772282,-0.146600315032072,
-0.144661579838321,-0.142583928024751,-0.139314981065769,-0.128824707791949,
-0.0985425252177895,-0.0750520070855559,-0.0747374496497559),
 .UNSPECIFIED.);
#1070=B_SPLINE_CURVE_WITH_KNOTS('',3,(#111092,#111093,#111094,#111095,#111096,
#111097,#111098,#111099,#111100,#111101,#111102,#111103,#111104,#111105,
#111106,#111107,#111108,#111109,#111110,#111111,#111112,#111113,#111114,
#111115,#111116,#111117,#111118,#111119,#111120,#111121,#111122,#111123,
#111124,#111125,#111126,#111127,#111128,#111129,#111130,#111131,#111132,
#111133,#111134,#111135,#111136,#111137,#111138,#111139,#111140,#111141,
#111142,#111143,#111144,#111145,#111146,#111147,#111148,#111149,#111150,
#111151,#111152,#111153,#111154,#111155,#111156,#111157,#111158,#111159,
#111160,#111161,#111162,#111163,#111164,#111165,#111166,#111167,#111168,
#111169,#111170,#111171,#111172,#111173,#111174,#111175,#111176,#111177,
#111178,#111179,#111180,#111181,#111182,#111183,#111184,#111185,#111186,
#111187,#111188,#111189,#111190,#111191,#111192,#111193,#111194,#111195,
#111196,#111197,#111198,#111199,#111200,#111201,#111202,#111203,#111204,
#111205,#111206,#111207,#111208,#111209,#111210,#111211,#111212,#111213,
#111214,#111215,#111216,#111217,#111218,#111219,#111220,#111221,#111222,
#111223,#111224,#111225,#111226,#111227,#111228,#111229,#111230,#111231,
#111232,#111233,#111234,#111235,#111236,#111237,#111238,#111239,#111240,
#111241,#111242,#111243,#111244,#111245,#111246,#111247,#111248,#111249,
#111250,#111251,#111252,#111253,#111254,#111255,#111256,#111257,#111258,
#111259,#111260,#111261,#111262,#111263,#111264,#111265,#111266,#111267,
#111268,#111269,#111270,#111271,#111272,#111273,#111274,#111275,#111276,
#111277,#111278,#111279,#111280,#111281,#111282,#111283,#111284,#111285,
#111286,#111287,#111288,#111289,#111290,#111291,#111292,#111293,#111294,
#111295,#111296,#111297,#111298,#111299,#111300,#111301,#111302,#111303,
#111304,#111305,#111306,#111307,#111308,#111309,#111310,#111311,#111312,
#111313,#111314,#111315,#111316,#111317,#111318,#111319,#111320,#111321,
#111322,#111323,#111324,#111325),.UNSPECIFIED.,.F.,.F.,(4,2,2,2,2,2,2,2,
2,2,2,2,2,2,2,2,2,2,2,2,2,2,2,2,2,2,2,2,2,2,2,2,2,2,2,2,2,2,2,2,2,2,2,2,
2,2,2,2,2,2,2,2,2,2,2,2,2,2,2,2,2,2,2,2,2,2,2,2,2,2,2,2,2,2,2,2,2,2,2,2,
2,2,2,2,2,2,2,2,2,2,2,2,2,2,2,2,2,2,2,2,2,2,2,2,2,2,2,2,2,2,2,2,2,2,2,2,
4),(-2.59315592110003,-2.59007760746276,-2.58078442575993,-2.57864192938728,
-2.57741401594,-2.57633919268755,-2.57495057949168,-2.57203620779358,-2.54225933787784,
-2.49161915788067,-2.48229151674428,-2.47774090940545,-2.47500323237432,
-2.47251935567029,-2.47064334858746,-2.46881679266551,-2.46627505840282,
-2.45963438585243,-2.40384856483129,-2.37977478395088,-2.36894861241379,
-2.36670457236547,-2.36545436799998,-2.3643824763686,-2.36302655672008,
-2.3608812914899,-2.3498481993763,-2.29862656964715,-2.26992243674973,-2.26348946250616,
-2.26078097146617,-2.25881939093963,-2.25702685582208,-2.25416198731251,
-2.24727744883033,-2.19421481901948,-2.16830142125363,-2.1569928671498,
-2.15472038807679,-2.15346400985927,-2.15239273879776,-2.15104513417737,
-2.14842386474133,-2.1323851049409,-2.127067161605,-2.11250735298119,-2.07961709049668,
-2.06305107213864,-2.05273920487412,-2.04949043458139,-2.04741712304519,
-2.0454764891654,-2.04293542792708,-2.03864073343987,-2.00353420408067,
-1.95464848169311,-1.94485971866109,-1.94268234715487,-1.94144672193535,
-1.94037303818875,-1.93899622349874,-1.93614245724537,-1.91343293577874,
-1.87271723892081,-1.84567967566739,-1.83944821448597,-1.83677396459371,
-1.83481838483426,-1.83301823941712,-1.83011233514104,-1.82298134565623,
-1.77424411226903,-1.73505279865021,-1.73147806748382,-1.72996904413746,
-1.72887687769649,-1.72785089466849,-1.72610769613703,-1.72137471656642,
-1.68178411444338,-1.63388987192041,-1.62749309716374,-1.62479052636968,
-1.62282983556348,-1.62103577072735,-1.61816334851162,-1.6112341799604,
-1.55875566853387,-1.53242878829024,-1.52101504518211,-1.518736407992,-1.51747862383898,
-1.51640745066291,-1.51506158912328,-1.51244824797811,-1.4965684694718,
-1.49069771123085,-1.4466670366256,-1.4281081624543,-1.41691845725991,-1.41357286267423,
-1.41147833616775,-1.40954560827383,-1.40705404740345,-1.4029285442078,
-1.37574263767364,-1.33373204800133,-1.32763515029272,-1.30978755198806,
-1.30709916585634,-1.30573723665793,-1.30466495507299,-1.30341928550094,
-1.3011958620241,-1.29070305466864,-1.26784055931316,-1.25960929803069),
 .UNSPECIFIED.);
#1071=B_SPLINE_CURVE_WITH_KNOTS('',3,(#111331,#111332,#111333,#111334,#111335,
#111336,#111337,#111338,#111339,#111340,#111341,#111342,#111343,#111344,
#111345,#111346,#111347,#111348,#111349,#111350,#111351,#111352,#111353,
#111354,#111355,#111356,#111357,#111358,#111359,#111360,#111361,#111362,
#111363,#111364,#111365,#111366,#111367,#111368,#111369,#111370,#111371,
#111372,#111373,#111374,#111375,#111376,#111377,#111378,#111379,#111380,
#111381,#111382,#111383,#111384,#111385,#111386,#111387,#111388,#111389,
#111390,#111391,#111392,#111393,#111394,#111395,#111396,#111397,#111398,
#111399,#111400,#111401,#111402,#111403,#111404,#111405,#111406,#111407,
#111408,#111409,#111410,#111411,#111412,#111413,#111414,#111415,#111416,
#111417,#111418,#111419,#111420,#111421,#111422,#111423,#111424,#111425,
#111426,#111427,#111428,#111429,#111430,#111431,#111432,#111433,#111434,
#111435,#111436),.UNSPECIFIED.,.F.,.F.,(4,3,3,3,3,3,3,3,3,3,3,3,3,3,3,3,
3,3,3,3,3,3,3,3,3,3,3,3,3,3,3,3,3,3,3,4),(-3.49054215479303,-3.38888735076487,
-3.28714626812733,-3.1853636260202,-3.08340269581344,-2.99650934988562,
-2.89298838415396,-2.78961842057155,-2.68636679313983,-2.58317880759896,
-2.48002064176422,-2.37685851496102,-2.27358841489215,-2.17026119505921,
-2.0667513667292,-1.99767289992375,-1.89536901188922,-1.79321917542624,
-1.69118674247088,-1.58921701577402,-1.48727463022104,-1.38532426116751,
-1.28325154596753,-1.18111583450429,-1.07877443242786,-0.998836449961874,
-0.892563151715311,-0.780992757750897,-0.67507278596415,-0.569252409114429,
-0.463503885892151,-0.35779956469349,-0.252082102978442,-0.14635955384072,
-0.0405640348441946,0.),.UNSPECIFIED.);
#1072=B_SPLINE_CURVE_WITH_KNOTS('',3,(#111439,#111440,#111441,#111442,#111443,
#111444,#111445,#111446,#111447,#111448,#111449,#111450,#111451,#111452,
#111453,#111454,#111455,#111456,#111457,#111458,#111459,#111460,#111461,
#111462,#111463,#111464,#111465,#111466,#111467,#111468,#111469,#111470,
#111471,#111472,#111473,#111474,#111475,#111476,#111477,#111478,#111479,
#111480,#111481,#111482,#111483,#111484,#111485,#111486,#111487,#111488,
#111489,#111490,#111491,#111492,#111493,#111494,#111495,#111496,#111497,
#111498,#111499,#111500,#111501,#111502,#111503,#111504,#111505,#111506,
#111507,#111508,#111509,#111510,#111511,#111512,#111513,#111514,#111515,
#111516,#111517,#111518,#111519,#111520,#111521,#111522,#111523,#111524,
#111525,#111526,#111527,#111528,#111529,#111530,#111531,#111532,#111533,
#111534,#111535,#111536,#111537,#111538,#111539,#111540,#111541,#111542,
#111543,#111544,#111545,#111546,#111547,#111548,#111549,#111550,#111551,
#111552,#111553,#111554,#111555,#111556,#111557,#111558,#111559,#111560,
#111561,#111562,#111563,#111564,#111565,#111566,#111567,#111568,#111569,
#111570,#111571,#111572,#111573,#111574,#111575,#111576,#111577,#111578,
#111579,#111580,#111581,#111582,#111583,#111584,#111585,#111586,#111587,
#111588,#111589,#111590,#111591,#111592,#111593,#111594,#111595,#111596,
#111597,#111598),.UNSPECIFIED.,.F.,.F.,(4,3,3,3,3,3,3,3,3,3,3,3,3,3,3,3,
3,3,3,3,3,3,3,3,3,3,3,3,3,3,3,3,3,3,3,3,3,3,3,3,3,3,3,3,3,3,3,3,3,3,3,3,
3,4),(2.00878451764821,2.1121039127969,2.21526989698106,2.31831446525083,
2.42129383098608,2.52424213980843,2.62719349431524,2.73024965054137,2.83336280284649,
2.93665222006088,2.99650934988562,3.10008230986107,3.20350557536155,3.30681224772107,
3.41005632831867,3.51327157245742,3.61649169494131,3.71982084946884,3.82320780718046,
3.92677785652894,3.9953457998475,4.09860812441836,4.20171508638263,4.30469852295221,
4.40761526975679,4.51049956061297,4.61338558491661,4.71637810302106,4.81942648355174,
4.92265858166651,4.99418224980938,5.09760358352984,5.20087156240149,5.30401824170998,
5.40709952008126,5.51014939511656,5.61320182122765,5.71636085636681,5.81957608032992,
5.92297369428319,5.99301869977126,6.09643423755246,6.19969678686738,6.30283861434794,
6.40591539958103,6.50896114779528,6.61200982139887,6.71516571129326,6.81837812515211,
6.92177350497573,6.99185514973313,7.09672279125044,7.20139613948791,7.24304105038295),
 .UNSPECIFIED.);
#1073=B_SPLINE_CURVE_WITH_KNOTS('',3,(#111601,#111602,#111603,#111604,#111605,
#111606,#111607,#111608,#111609,#111610,#111611,#111612,#111613),
 .UNSPECIFIED.,.F.,.F.,(4,3,3,3,4),(7.24304105038295,7.3475229962934,7.45192126808273,
7.55626822218831,7.5925217232362),.UNSPECIFIED.);
#1074=B_SPLINE_CURVE_WITH_KNOTS('',3,(#111614,#111615,#111616,#111617,#111618,
#111619,#111620,#111621,#111622,#111623,#111624,#111625,#111626,#111627,
#111628,#111629,#111630,#111631,#111632,#111633,#111634,#111635,#111636,
#111637,#111638,#111639,#111640,#111641,#111642,#111643,#111644,#111645,
#111646,#111647,#111648,#111649,#111650,#111651,#111652,#111653,#111654,
#111655,#111656,#111657,#111658,#111659,#111660,#111661,#111662,#111663,
#111664,#111665,#111666,#111667,#111668,#111669,#111670,#111671,#111672,
#111673,#111674,#111675,#111676,#111677,#111678,#111679,#111680,#111681,
#111682,#111683,#111684,#111685,#111686,#111687,#111688,#111689,#111690,
#111691,#111692,#111693,#111694,#111695,#111696,#111697,#111698,#111699,
#111700,#111701,#111702,#111703,#111704,#111705,#111706,#111707,#111708,
#111709,#111710,#111711,#111712,#111713,#111714,#111715,#111716,#111717,
#111718,#111719,#111720,#111721,#111722,#111723,#111724,#111725,#111726,
#111727,#111728,#111729,#111730,#111731,#111732,#111733,#111734,#111735,
#111736,#111737,#111738,#111739,#111740,#111741,#111742,#111743,#111744,
#111745,#111746,#111747,#111748,#111749,#111750,#111751,#111752,#111753,
#111754,#111755,#111756,#111757,#111758,#111759,#111760,#111761,#111762,
#111763,#111764,#111765,#111766,#111767,#111768,#111769,#111770,#111771,
#111772,#111773,#111774,#111775,#111776,#111777,#111778,#111779,#111780,
#111781,#111782,#111783,#111784,#111785,#111786,#111787,#111788,#111789,
#111790,#111791,#111792,#111793,#111794,#111795,#111796,#111797,#111798,
#111799,#111800,#111801,#111802,#111803,#111804,#111805,#111806,#111807,
#111808,#111809,#111810,#111811,#111812,#111813,#111814,#111815,#111816,
#111817,#111818,#111819,#111820,#111821,#111822,#111823,#111824,#111825,
#111826,#111827,#111828,#111829,#111830,#111831,#111832,#111833,#111834,
#111835,#111836,#111837),.UNSPECIFIED.,.F.,.F.,(4,2,2,2,2,2,2,2,2,2,2,2,
2,2,2,2,2,2,2,2,2,2,2,2,2,2,2,2,2,2,2,2,2,2,2,2,2,2,2,2,2,2,2,2,2,2,2,2,
2,2,2,2,2,2,2,2,2,2,2,2,2,2,2,2,2,2,2,2,2,2,2,2,2,2,2,2,2,2,2,2,2,2,2,2,
2,2,2,2,2,2,2,2,2,2,2,2,2,2,2,2,2,2,2,2,2,2,2,2,2,2,2,4),(-2.66727271147711,
-2.64514416123945,-2.59598682591251,-2.58660188532894,-2.58445439068241,
-2.58322622212268,-2.58215204826259,-2.58076604165038,-2.57786525834857,
-2.55097420357146,-2.51353771549261,-2.49429289537454,-2.48669443218254,
-2.48276636104382,-2.47945649826737,-2.47740192605286,-2.47547608342467,
-2.47299780604071,-2.46900881820271,-2.44540125182709,-2.39836981398955,
-2.38274909190571,-2.37453345221375,-2.37247353224399,-2.3712634653851,
-2.37018463046746,-2.36878790365098,-2.36645716905911,-2.35190421798962,
-2.34958113653479,-2.30363635510011,-2.27573127058486,-2.26939428504012,
-2.26670206614296,-2.26474341268377,-2.2629474242732,-2.26006362258563,
-2.2530643410738,-2.20164290380157,-2.174559750452,-2.16295806679369,-2.16066914658454,
-2.15940927313382,-2.15833842129164,-2.15699565879203,-2.15439636277061,
-2.13885999261317,-2.13223205772158,-2.11842240488002,-2.08554052236304,
-2.06898364824746,-2.0586762010965,-2.05542820156501,-2.05335523703073,
-2.05141482761761,-2.04887391745638,-2.04457916477255,-2.00944108908087,
-1.96049945514058,-1.95078674134142,-1.94861477560486,-1.94738044024498,
-1.94630663183684,-1.94492809590307,-1.94206564076842,-1.918706272745,-1.9064090561897,
-1.87354001080172,-1.85700030741615,-1.84670002718578,-1.84345234324541,
-1.84137910534026,-1.8394381038791,-1.83689592979739,-1.83259793217183,
-1.79725558910473,-1.74808177107833,-1.73876433087334,-1.73661980194068,
-1.73539129338086,-1.7343163695614,-1.73292814162882,-1.73001627459185,
-1.69798300408521,-1.66507278295209,-1.64624531853499,-1.6387608006613,
-1.6331384018191,-1.63057275744381,-1.62863505227293,-1.62680647601108,
-1.62425779356639,-1.61757401128421,-1.56218086420771,-1.53783841722789,
-1.52693939559833,-1.52469073589719,-1.52343941933517,-1.52236748220644,
-1.52101266770936,-1.51835847063183,-1.50147594892666,-1.482688240376,-1.44972214359721,
-1.43306884299333,-1.42271704818392,-1.41946333617731,-1.41738870063118,
-1.41544811106488,-1.41290895773657,-1.40862162865882,-1.40825517075566),
 .UNSPECIFIED.);
#1075=B_SPLINE_CURVE_WITH_KNOTS('',3,(#111839,#111840,#111841,#111842,#111843,
#111844,#111845,#111846,#111847,#111848,#111849,#111850,#111851,#111852,
#111853,#111854,#111855,#111856,#111857,#111858,#111859,#111860,#111861,
#111862,#111863,#111864,#111865,#111866,#111867,#111868,#111869,#111870,
#111871,#111872,#111873,#111874,#111875,#111876,#111877,#111878,#111879,
#111880,#111881,#111882,#111883,#111884,#111885,#111886,#111887,#111888,
#111889,#111890,#111891,#111892,#111893,#111894,#111895,#111896,#111897,
#111898,#111899,#111900,#111901,#111902,#111903,#111904,#111905,#111906,
#111907,#111908,#111909,#111910,#111911,#111912,#111913,#111914,#111915,
#111916,#111917,#111918,#111919,#111920,#111921,#111922,#111923,#111924,
#111925,#111926,#111927,#111928,#111929,#111930,#111931,#111932,#111933,
#111934,#111935,#111936,#111937,#111938,#111939,#111940,#111941,#111942,
#111943,#111944,#111945,#111946,#111947,#111948,#111949,#111950,#111951,
#111952,#111953,#111954,#111955,#111956,#111957,#111958,#111959,#111960,
#111961,#111962,#111963,#111964,#111965,#111966,#111967,#111968,#111969,
#111970,#111971,#111972,#111973,#111974,#111975,#111976,#111977,#111978,
#111979,#111980,#111981,#111982,#111983,#111984,#111985,#111986,#111987,
#111988,#111989,#111990,#111991,#111992,#111993,#111994,#111995,#111996,
#111997,#111998,#111999,#112000,#112001,#112002,#112003,#112004,#112005,
#112006,#112007,#112008,#112009,#112010,#112011,#112012,#112013,#112014,
#112015,#112016,#112017,#112018,#112019,#112020,#112021,#112022,#112023,
#112024,#112025,#112026,#112027,#112028,#112029,#112030,#112031,#112032,
#112033,#112034,#112035,#112036,#112037,#112038,#112039,#112040,#112041,
#112042,#112043,#112044,#112045,#112046,#112047,#112048,#112049,#112050,
#112051,#112052,#112053,#112054,#112055,#112056,#112057,#112058,#112059,
#112060),.UNSPECIFIED.,.F.,.F.,(4,2,2,2,2,2,2,2,2,2,2,2,2,2,2,2,2,2,2,2,
2,2,2,2,2,2,2,2,2,2,2,2,2,2,2,2,2,2,2,2,2,2,2,2,2,2,2,2,2,2,2,2,2,2,2,2,
2,2,2,2,2,2,2,2,2,2,2,2,2,2,2,2,2,2,2,2,2,2,2,2,2,2,2,2,2,2,2,2,2,2,2,2,
2,2,2,2,2,2,2,2,2,2,2,2,2,2,2,2,2,2,4),(-1.25960929803069,-1.21011174059313,
-1.20367847070001,-1.20117010943763,-1.19935225139578,-1.19740896028293,
-1.19480675371619,-1.18898303134276,-1.16514968953682,-1.11614974413865,
-1.09779133614114,-1.09505199506547,-1.09369780555932,-1.09262570481289,
-1.091373288173,-1.0891211906243,-1.07817670271,-1.0536606039483,-0.998557337097207,
-0.99185015018964,-0.989297536679468,-0.987467670152941,-0.985529994360003,
-0.982966737023876,-0.977358997910008,-0.929075022523474,-0.888723650897612,
-0.884011293331561,-0.882271319328065,-0.881246034995388,-0.880154599411069,
-0.878645304763367,-0.875062783457867,-0.87003765954688,-0.856213798932361,
-0.833862851050275,-0.787184857092799,-0.779989353322992,-0.77707435160675,
-0.775273835415769,-0.773322011139474,-0.770660371509933,-0.764492312114575,
-0.737949751057634,-0.698620981785537,-0.687287703556983,-0.673503625815556,
-0.671211226208082,-0.669826491416476,-0.668750040710085,-0.667534910834848,
-0.665449578878858,-0.656908102706735,-0.640347757197037,-0.598278136195905,
-0.57109945539481,-0.566971932881447,-0.564479109437179,-0.562545367777876,
-0.560449702725794,-0.557102184858802,-0.545904431502816,-0.527329184645362,
-0.484805743872738,-0.462028553407037,-0.459170664799327,-0.457792004451033,
-0.456715739894236,-0.45547476300475,-0.453287175566931,-0.443435343816671,
-0.394232923641606,-0.359839149025425,-0.355551442270918,-0.353009445992766,
-0.35106507330854,-0.348984785261022,-0.345718755854318,-0.335297069174024,
-0.318505453670392,-0.258883112535898,-0.249294109526251,-0.247244777885605,
-0.245918161908627,-0.244851122932402,-0.24384140172536,-0.241869006075161,
-0.234450995222338,-0.220917592501162,-0.192337588586147,-0.147271549613432,
-0.143024726566531,-0.140506655582846,-0.138580647851886,-0.136520206534398,
-0.133286041550045,-0.122977073904068,-0.106384488990819,-0.0845184569141308,
-0.0739378345267708,-0.0616381299481483,-0.0559579040156458,-0.0377855980021243,
-0.0350634423940383,-0.0337175280400151,-0.0326484421208826,-0.0316335711034375,
-0.030396079803991,-0.0285521106333106,-0.021532695795065,-0.00065555409686486),
 .UNSPECIFIED.);
#1076=B_SPLINE_CURVE_WITH_KNOTS('',3,(#112061,#112062,#112063,#112064,#112065,
#112066,#112067,#112068,#112069,#112070,#112071,#112072,#112073),
 .UNSPECIFIED.,.F.,.F.,(4,3,3,3,4),(-3.84103903298818,-3.73916989819696,
-3.63740764530368,-3.53571860707482,-3.49054215479303),.UNSPECIFIED.);
#1077=B_SPLINE_CURVE_WITH_KNOTS('',3,(#112076,#112077,#112078,#112079,#112080,
#112081,#112082,#112083,#112084,#112085,#112086,#112087,#112088),
 .UNSPECIFIED.,.F.,.F.,(4,3,3,3,4),(7.24304095782437,7.34752291252988,7.45192119316322,
7.55626815616017,7.5925217232362),.UNSPECIFIED.);
#1078=B_SPLINE_CURVE_WITH_KNOTS('',3,(#112089,#112090,#112091,#112092,#112093,
#112094,#112095,#112096,#112097,#112098,#112099,#112100,#112101,#112102,
#112103,#112104,#112105,#112106,#112107,#112108,#112109,#112110,#112111,
#112112,#112113,#112114,#112115,#112116,#112117,#112118,#112119,#112120,
#112121,#112122,#112123,#112124,#112125,#112126,#112127,#112128,#112129,
#112130,#112131,#112132,#112133,#112134,#112135,#112136,#112137,#112138,
#112139,#112140,#112141,#112142,#112143,#112144,#112145,#112146,#112147,
#112148,#112149,#112150,#112151,#112152,#112153,#112154,#112155,#112156,
#112157,#112158,#112159,#112160,#112161,#112162,#112163,#112164,#112165,
#112166,#112167,#112168,#112169,#112170,#112171,#112172,#112173,#112174,
#112175,#112176,#112177,#112178,#112179,#112180,#112181,#112182,#112183,
#112184,#112185,#112186,#112187,#112188,#112189,#112190,#112191,#112192,
#112193,#112194,#112195,#112196,#112197,#112198,#112199,#112200,#112201,
#112202,#112203,#112204,#112205,#112206,#112207,#112208,#112209,#112210,
#112211,#112212,#112213,#112214,#112215,#112216,#112217,#112218,#112219,
#112220,#112221,#112222,#112223,#112224,#112225,#112226,#112227,#112228,
#112229,#112230,#112231,#112232,#112233,#112234,#112235,#112236,#112237,
#112238,#112239,#112240,#112241,#112242,#112243,#112244,#112245,#112246,
#112247,#112248,#112249,#112250,#112251,#112252,#112253,#112254,#112255,
#112256,#112257,#112258,#112259,#112260,#112261,#112262,#112263,#112264,
#112265,#112266,#112267,#112268,#112269,#112270,#112271,#112272,#112273,
#112274,#112275,#112276,#112277,#112278,#112279,#112280,#112281,#112282,
#112283,#112284,#112285,#112286,#112287,#112288,#112289,#112290,#112291,
#112292,#112293,#112294,#112295,#112296,#112297,#112298,#112299,#112300,
#112301,#112302,#112303,#112304,#112305,#112306,#112307,#112308,#112309,
#112310,#112311,#112312,#112313,#112314),.UNSPECIFIED.,.F.,.F.,(4,2,2,2,
2,2,2,2,2,2,2,2,2,2,2,2,2,2,2,2,2,2,2,2,2,2,2,2,2,2,2,2,2,2,2,2,2,2,2,2,
2,2,2,2,2,2,2,2,2,2,2,2,2,2,2,2,2,2,2,2,2,2,2,2,2,2,2,2,2,2,2,2,2,2,2,2,
2,2,2,2,2,2,2,2,2,2,2,2,2,2,2,2,2,2,2,2,2,2,2,2,2,2,2,2,2,2,2,2,2,2,2,2,
4),(-2.66738008698545,-2.62224783784958,-2.59781807626665,-2.58689866123443,
-2.58465077822854,-2.58340061958436,-2.58232936394948,-2.5809754340121,
-2.57823682703122,-2.55989579598849,-2.54256186398593,-2.50963546001051,
-2.49302151413064,-2.48615785461855,-2.48250535135525,-2.47938648970499,
-2.47737576448748,-2.47543621773921,-2.47290497400306,-2.46864554443795,
-2.43625798350028,-2.38684716722421,-2.3750771819673,-2.37277788668897,
-2.371515230832,-2.37044400533806,-2.36910315768299,-2.36700741861124,-2.3567449683609,
-2.35162580739283,-2.34970817795153,-2.30375081737001,-2.27584422957403,
-2.26950703470382,-2.26681476519162,-2.26485608899408,-2.26306008949113,
-2.26017629141725,-2.25317712794255,-2.20175227992819,-2.1746709946617,
-2.16306972535565,-2.16078081288259,-2.1595209339716,-2.1584500716418,-2.15710728856331,
-2.1545079310582,-2.13897054293179,-2.13234428594965,-2.11853372607665,
-2.08565153311177,-2.06909449796636,-2.05878695179806,-2.05553892165284,
-2.05346593771655,-2.05152551023676,-2.04898457655228,-2.04468978440395,
-2.00955141633932,-1.96060940061397,-1.950896509287,-1.94872451732727,-1.94749016914898,
-1.94641635098428,-1.94503780430775,-1.9421753328758,-1.91881626262359,
-1.9065184180079,-1.87364906551616,-1.85710920486868,-1.84680882756439,
-1.84356111345625,-1.84148785639893,-1.83954683708113,-1.83700463971943,
-1.8327066029785,-1.79736397701867,-1.74818967157994,-1.73887213386421,
-1.73672758436278,-1.73549906432215,-1.73442413061742,-1.73303589015582,
-1.73012399776097,-1.69809709466842,-1.66517975028743,-1.64635221385029,
-1.63886765464738,-1.63324522036375,-1.63067955529907,-1.62874183265477,
-1.62691323854142,-1.62436452902093,-1.61768066234483,-1.56228724285179,
-1.53794441598955,-1.52704525222948,-1.52479656921338,-1.5235452405122,
-1.52247329349964,-1.52111846716453,-1.5184642488387,-1.50158165907637,
-1.48279369110174,-1.44982728879555,-1.43317383267406,-1.42282194145276,
-1.41956819924802,-1.41749354447039,-1.41555293693074,-1.41301376010656,
-1.40872639140123,-1.40835994883514),.UNSPECIFIED.);
#1079=B_SPLINE_CURVE_WITH_KNOTS('',3,(#112316,#112317,#112318,#112319,#112320,
#112321,#112322,#112323,#112324,#112325,#112326,#112327,#112328,#112329,
#112330,#112331,#112332,#112333,#112334,#112335,#112336,#112337,#112338,
#112339,#112340,#112341,#112342,#112343,#112344,#112345,#112346,#112347,
#112348,#112349,#112350,#112351,#112352,#112353,#112354,#112355,#112356,
#112357,#112358,#112359,#112360,#112361,#112362,#112363,#112364,#112365,
#112366,#112367,#112368,#112369,#112370,#112371,#112372,#112373,#112374,
#112375,#112376,#112377,#112378,#112379,#112380,#112381,#112382,#112383,
#112384,#112385,#112386,#112387,#112388,#112389,#112390,#112391,#112392,
#112393,#112394,#112395,#112396,#112397,#112398,#112399,#112400,#112401,
#112402,#112403,#112404,#112405,#112406,#112407,#112408,#112409,#112410,
#112411,#112412,#112413,#112414,#112415,#112416,#112417,#112418,#112419,
#112420,#112421,#112422,#112423,#112424,#112425,#112426,#112427,#112428,
#112429,#112430,#112431,#112432,#112433,#112434,#112435,#112436,#112437,
#112438,#112439,#112440,#112441,#112442,#112443,#112444,#112445,#112446,
#112447,#112448,#112449,#112450,#112451,#112452,#112453,#112454,#112455,
#112456,#112457,#112458,#112459,#112460,#112461,#112462,#112463,#112464,
#112465,#112466,#112467,#112468,#112469,#112470,#112471,#112472,#112473,
#112474,#112475,#112476,#112477,#112478,#112479,#112480,#112481,#112482,
#112483,#112484,#112485,#112486,#112487,#112488,#112489,#112490,#112491,
#112492,#112493,#112494,#112495,#112496,#112497,#112498,#112499,#112500,
#112501,#112502,#112503,#112504,#112505,#112506,#112507,#112508,#112509,
#112510,#112511,#112512,#112513,#112514,#112515,#112516,#112517,#112518,
#112519,#112520,#112521,#112522,#112523,#112524,#112525,#112526,#112527,
#112528,#112529,#112530,#112531,#112532,#112533,#112534,#112535,#112536,
#112537),.UNSPECIFIED.,.F.,.F.,(4,2,2,2,2,2,2,2,2,2,2,2,2,2,2,2,2,2,2,2,
2,2,2,2,2,2,2,2,2,2,2,2,2,2,2,2,2,2,2,2,2,2,2,2,2,2,2,2,2,2,2,2,2,2,2,2,
2,2,2,2,2,2,2,2,2,2,2,2,2,2,2,2,2,2,2,2,2,2,2,2,2,2,2,2,2,2,2,2,2,2,2,2,
2,2,2,2,2,2,2,2,2,2,2,2,2,2,2,2,2,2,4),(-1.2596092791427,-1.21011169664944,
-1.20367842859327,-1.20117006796674,-1.19935221036289,-1.19740891969948,
-1.19480671370743,-1.1889829925253,-1.16514965425979,-1.11614969218952,
-1.09779132074701,-1.09505198071949,-1.09369779134588,-1.09262569009982,
-1.09137327188847,-1.0891211707322,-1.07817664855281,-1.05366042450533,
-0.998557438618785,-0.991850234273926,-0.989297617185117,-0.987467749012962,
-0.985530072311542,-0.982966815170316,-0.977359082047891,-0.929076048470101,
-0.888723759846889,-0.884011357367577,-0.882271376440202,-0.881246090678849,
-0.880154657239091,-0.878645369768322,-0.87506288280695,-0.870037819142832,
-0.856214195879545,-0.833860460614285,-0.787184959555151,-0.779989405419897,
-0.777074397744445,-0.775273882355138,-0.77332206248597,-0.770660435232421,
-0.764492433475752,-0.737950307557521,-0.698623437672005,-0.68728966454219,
-0.673503806106148,-0.671211322848425,-0.669826564557874,-0.668750112408046,
-0.667534999889146,-0.665449740786321,-0.656909155741711,-0.640351409192942,
-0.598279168069409,-0.571099321214126,-0.566971768417946,-0.564478936343208,
-0.562545193753715,-0.560449533462879,-0.557102035727017,-0.545904467008763,
-0.527329643544558,-0.484795377006182,-0.462028090530099,-0.459170447779128,
-0.457791834481783,-0.456715570669755,-0.455474553101724,-0.453286801311886,
-0.443432679424966,-0.394231696149154,-0.359839482001392,-0.355551793568,
-0.353009797948434,-0.351065419758364,-0.348985119919028,-0.345719059516173,
-0.335297165786895,-0.318505114312126,-0.258883412648892,-0.249294304900512,
-0.247244964361322,-0.24591834496186,-0.244851306982384,-0.243841592595941,
-0.241869215319139,-0.23445132044746,-0.220918198218288,-0.192338068365553,
-0.147271574269591,-0.143024776704226,-0.140506721051313,-0.138580725286331,
-0.136520297076973,-0.133286153483837,-0.122977264284867,-0.106384825868077,
-0.0845186660431512,-0.0739384345445597,-0.0616384513993995,-0.0559535320440041,
-0.0377853867776285,-0.0350633807398456,-0.0337175017363041,-0.0326484251826848,
-0.0316335581109729,-0.030396058734142,-0.0285520611649711,-0.0215326044775512,
-0.00065556807277999),.UNSPECIFIED.);
#1080=B_SPLINE_CURVE_WITH_KNOTS('',3,(#112538,#112539,#112540,#112541,#112542,
#112543,#112544,#112545,#112546,#112547,#112548,#112549,#112550),
 .UNSPECIFIED.,.F.,.F.,(4,3,3,3,4),(-3.8410390329882,-3.7391698932069,-3.63740763660875,
-3.53571859652656,-3.4905420523601),.UNSPECIFIED.);
#1081=B_SPLINE_CURVE_WITH_KNOTS('',3,(#112553,#112554,#112555,#112556,#112557,
#112558,#112559,#112560,#112561,#112562,#112563,#112564,#112565),
 .UNSPECIFIED.,.F.,.F.,(4,3,3,3,4),(7.2430409600995,7.34752291120672,7.45192118821202,
7.55626814755434,7.5925217232362),.UNSPECIFIED.);
#1082=B_SPLINE_CURVE_WITH_KNOTS('',3,(#112566,#112567,#112568,#112569,#112570,
#112571,#112572,#112573,#112574,#112575,#112576,#112577,#112578,#112579,
#112580,#112581,#112582,#112583,#112584,#112585,#112586,#112587,#112588,
#112589,#112590,#112591,#112592,#112593,#112594,#112595,#112596,#112597,
#112598,#112599,#112600,#112601,#112602,#112603,#112604,#112605,#112606,
#112607,#112608,#112609,#112610,#112611,#112612,#112613,#112614,#112615,
#112616,#112617,#112618,#112619,#112620,#112621,#112622,#112623,#112624,
#112625,#112626,#112627,#112628,#112629,#112630,#112631,#112632,#112633,
#112634,#112635,#112636,#112637,#112638,#112639,#112640,#112641,#112642,
#112643,#112644,#112645,#112646,#112647,#112648,#112649,#112650,#112651,
#112652,#112653,#112654,#112655,#112656,#112657,#112658,#112659,#112660,
#112661,#112662,#112663,#112664,#112665,#112666,#112667,#112668,#112669,
#112670,#112671,#112672,#112673,#112674,#112675,#112676,#112677,#112678,
#112679,#112680,#112681,#112682,#112683,#112684,#112685,#112686,#112687,
#112688,#112689,#112690,#112691,#112692,#112693,#112694,#112695,#112696,
#112697,#112698,#112699,#112700,#112701,#112702,#112703,#112704,#112705,
#112706,#112707,#112708,#112709,#112710,#112711,#112712,#112713,#112714,
#112715,#112716,#112717,#112718,#112719,#112720,#112721,#112722,#112723,
#112724,#112725,#112726,#112727,#112728,#112729,#112730,#112731,#112732,
#112733,#112734,#112735,#112736,#112737,#112738,#112739,#112740,#112741,
#112742,#112743,#112744,#112745,#112746,#112747,#112748,#112749,#112750,
#112751,#112752,#112753,#112754,#112755,#112756,#112757,#112758,#112759,
#112760,#112761,#112762,#112763,#112764,#112765,#112766,#112767,#112768,
#112769,#112770,#112771,#112772,#112773,#112774,#112775,#112776,#112777,
#112778,#112779,#112780,#112781,#112782,#112783,#112784,#112785,#112786,
#112787,#112788,#112789,#112790,#112791),.UNSPECIFIED.,.F.,.F.,(4,2,2,2,
2,2,2,2,2,2,2,2,2,2,2,2,2,2,2,2,2,2,2,2,2,2,2,2,2,2,2,2,2,2,2,2,2,2,2,2,
2,2,2,2,2,2,2,2,2,2,2,2,2,2,2,2,2,2,2,2,2,2,2,2,2,2,2,2,2,2,2,2,2,2,2,2,
2,2,2,2,2,2,2,2,2,2,2,2,2,2,2,2,2,2,2,2,2,2,2,2,2,2,2,2,2,2,2,2,2,2,2,2,
4),(-2.66730687879803,-2.64516059795848,-2.59597250440395,-2.58663388874494,
-2.5844897853591,-2.58326240108112,-2.58218815896832,-2.58080107566422,
-2.57789455211048,-2.55020246391889,-2.51345475354417,-2.49429362638936,
-2.48671793935886,-2.48279836081912,-2.47949437709281,-2.47744121871936,
-2.47560711525565,-2.47317516578146,-2.46933881710637,-2.44888830435509,
-2.3998575173308,-2.3832044732505,-2.37463043778995,-2.37254157870367,-2.37132511676415,
-2.3702477505218,-2.368862206611,-2.36656943007814,-2.35280908560213,-2.35171480594859,
-2.34963344277311,-2.30368328812431,-2.27577856566349,-2.26944174036203,
-2.26674961218141,-2.26479103304299,-2.26299511854612,-2.26011144819991,
-2.2531125500284,-2.20169140113042,-2.17461056513675,-2.16300964613649,
-2.16072083305361,-2.15946101282519,-2.15839020276534,-2.15704748826761,
-2.15444827237636,-2.13891199681551,-2.13228535013131,-2.1184757802571,
-2.08559518754418,-2.0690389600921,-2.05873191624902,-2.05548404415292,
-2.05341116103188,-2.05147082788239,-2.04893001766635,-2.04463543408901,
-2.00949876012414,-1.96055909398235,-1.95084670976453,-1.94867482579937,
-1.94744053815821,-1.94636677209731,-1.94498829159577,-1.94212595516369,
-1.91876781382108,-1.90647077296417,-1.87360301875142,-1.8570639634473,
-1.84676408733396,-1.84351653107586,-1.84144337474289,-1.83950244969533,
-1.83696037575888,-1.83266254759222,-1.79732162117904,-1.7481497180924,
-1.73883263765423,-1.73668819264555,-1.73545973234315,-1.7343848508444,
-1.7329966777096,-1.73008492616404,-1.69805682769749,-1.66514389826425,
-1.64631723445147,-1.63883302738929,-1.63321085945028,-1.63064531779105,
-1.62870768911201,-1.62687918423403,-1.62433059999678,-1.6176470674001,
-1.5622562402909,-1.53791466010126,-1.52701604297646,-1.52476747025897,
-1.52351620259121,-1.52244430765029,-1.52108954685869,-1.51843545613556,
-1.50155365029971,-1.48276663059011,-1.44980183034579,-1.43314918401495,
-1.42279779605753,-1.41954421199193,-1.41746965803777,-1.41552914480069,
-1.41299009135711,-1.40870293095995,-1.40833650609706),.UNSPECIFIED.);
#1083=B_SPLINE_CURVE_WITH_KNOTS('',3,(#112793,#112794,#112795,#112796,#112797,
#112798,#112799,#112800,#112801,#112802,#112803,#112804,#112805,#112806,
#112807,#112808,#112809,#112810,#112811,#112812,#112813,#112814,#112815,
#112816,#112817,#112818,#112819,#112820,#112821,#112822,#112823,#112824,
#112825,#112826,#112827,#112828,#112829,#112830,#112831,#112832,#112833,
#112834,#112835,#112836,#112837,#112838,#112839,#112840,#112841,#112842,
#112843,#112844,#112845,#112846,#112847,#112848,#112849,#112850,#112851,
#112852,#112853,#112854,#112855,#112856,#112857,#112858,#112859,#112860,
#112861,#112862,#112863,#112864,#112865,#112866,#112867,#112868,#112869,
#112870,#112871,#112872,#112873,#112874,#112875,#112876,#112877,#112878,
#112879,#112880,#112881,#112882,#112883,#112884,#112885,#112886,#112887,
#112888,#112889,#112890,#112891,#112892,#112893,#112894,#112895,#112896,
#112897,#112898,#112899,#112900,#112901,#112902,#112903,#112904,#112905,
#112906,#112907,#112908,#112909,#112910,#112911,#112912,#112913,#112914,
#112915,#112916,#112917,#112918,#112919,#112920,#112921,#112922,#112923,
#112924,#112925,#112926,#112927,#112928,#112929,#112930,#112931,#112932,
#112933,#112934,#112935,#112936,#112937,#112938,#112939,#112940,#112941,
#112942,#112943,#112944,#112945,#112946,#112947,#112948,#112949,#112950,
#112951,#112952,#112953,#112954,#112955,#112956,#112957,#112958,#112959,
#112960,#112961,#112962,#112963,#112964,#112965,#112966,#112967,#112968,
#112969,#112970,#112971,#112972,#112973,#112974,#112975,#112976,#112977,
#112978,#112979,#112980,#112981,#112982,#112983,#112984,#112985,#112986,
#112987,#112988,#112989,#112990,#112991,#112992,#112993,#112994,#112995,
#112996,#112997,#112998,#112999,#113000,#113001,#113002,#113003,#113004,
#113005,#113006,#113007,#113008,#113009,#113010,#113011,#113012,#113013,
#113014),.UNSPECIFIED.,.F.,.F.,(4,2,2,2,2,2,2,2,2,2,2,2,2,2,2,2,2,2,2,2,
2,2,2,2,2,2,2,2,2,2,2,2,2,2,2,2,2,2,2,2,2,2,2,2,2,2,2,2,2,2,2,2,2,2,2,2,
2,2,2,2,2,2,2,2,2,2,2,2,2,2,2,2,2,2,2,2,2,2,2,2,2,2,2,2,2,2,2,2,2,2,2,2,
2,2,2,2,2,2,2,2,2,2,2,2,2,2,2,2,2,2,4),(-1.25960927882884,-1.21011169532823,
-1.20367842731546,-1.20117006670425,-1.19935220911066,-1.19740891845822,
-1.1948067124806,-1.18898299132885,-1.16514965315903,-1.11614969077259,
-1.09779132013028,-1.09505198012728,-1.09369779075751,-1.09262568950179,
-1.09137327125847,-1.08912117002723,-1.07817664712381,-1.05366042041119,
-0.998557440635837,-0.991850235923305,-0.989297618760896,-0.987467750555575,
-0.985530073836942,-0.982966816703447,-0.977359083717694,-0.929076070422091,
-0.888723762183214,-0.884011358744775,-0.882271377671097,-0.881246091880497,
-0.880154658488213,-0.878645371172887,-0.875062884953175,-0.870037822588928,
-0.85621420444147,-0.833860409293135,-0.787184961841286,-0.77998940663088,
-0.777074398830036,-0.775273883459694,-0.773322063687082,-0.770660436701997,
-0.764492436189761,-0.737950319646653,-0.698623490627323,-0.687289707791117,
-0.673503810242227,-0.671211325147951,-0.669826566341357,-0.668750114159319,
-0.667535002020493,-0.665449744515916,-0.656909179027754,-0.64035148951231,
-0.598279190791866,-0.571099318538436,-0.56697176508342,-0.564478932820849,
-0.562545190211058,-0.560449530023899,-0.557102032726576,-0.545904468030332,
-0.527329653789821,-0.484795151298745,-0.462028080676498,-0.45917044328081,
-0.457791831008699,-0.456715567213456,-0.455474548760424,-0.45328679339357,
-0.44343262163769,-0.394231669735219,-0.359839489357513,-0.355551801319755,
-0.353009805714651,-0.351065427406005,-0.348985127312124,-0.345719066239315,
-0.335297168033496,-0.318505107132256,-0.258883419254725,-0.249294309271303,
-0.247244968541648,-0.245918349068586,-0.24485131111036,-0.243841596870197,
-0.241869219986305,-0.234451327593885,-0.220918211360422,-0.192338078805669,
-0.147271574900182,-0.143024777879832,-0.140506722555446,-0.138580727046731,
-0.136520299117926,-0.133286155983296,-0.122977268470218,-0.106384833205498,
-0.0845186705986564,-0.0739384475260423,-0.0616384583542045,-0.0559534378375188,
-0.03778538222746,-0.0350633794114932,-0.0337175011687427,-0.0326484248162633,
-0.0316335578296692,-0.0303960582785997,-0.028552060096841,-0.0215326025070754,
-0.000655568373725938),.UNSPECIFIED.);
#1084=B_SPLINE_CURVE_WITH_KNOTS('',3,(#113015,#113016,#113017,#113018,#113019,
#113020,#113021,#113022,#113023,#113024,#113025,#113026,#113027),
 .UNSPECIFIED.,.F.,.F.,(4,3,3,3,4),(-3.84103903298819,-3.73916989309881,
-3.63740763642035,-3.53571859629846,-3.4905420525369),.UNSPECIFIED.);
#1085=B_SPLINE_CURVE_WITH_KNOTS('',3,(#113030,#113031,#113032,#113033,#113034,
#113035,#113036,#113037,#113038,#113039,#113040,#113041,#113042),
 .UNSPECIFIED.,.F.,.F.,(4,3,3,3,4),(7.24304101724442,7.34752294213327,7.45192119271409,
7.5562681254478,7.5925217232362),.UNSPECIFIED.);
#1086=B_SPLINE_CURVE_WITH_KNOTS('',3,(#113043,#113044,#113045,#113046,#113047,
#113048,#113049,#113050,#113051,#113052,#113053,#113054,#113055,#113056,
#113057,#113058,#113059,#113060,#113061,#113062,#113063,#113064,#113065,
#113066,#113067,#113068,#113069,#113070,#113071,#113072,#113073,#113074,
#113075,#113076,#113077,#113078,#113079,#113080,#113081,#113082,#113083,
#113084,#113085,#113086,#113087,#113088,#113089,#113090,#113091,#113092,
#113093,#113094,#113095,#113096,#113097,#113098,#113099,#113100,#113101,
#113102,#113103,#113104,#113105,#113106,#113107,#113108,#113109,#113110,
#113111,#113112,#113113,#113114,#113115,#113116,#113117,#113118,#113119,
#113120,#113121,#113122,#113123,#113124,#113125,#113126,#113127,#113128,
#113129,#113130,#113131,#113132,#113133,#113134,#113135,#113136,#113137,
#113138,#113139,#113140,#113141,#113142,#113143,#113144,#113145,#113146,
#113147,#113148,#113149,#113150,#113151,#113152,#113153,#113154,#113155,
#113156,#113157,#113158,#113159,#113160,#113161,#113162,#113163,#113164,
#113165,#113166,#113167,#113168,#113169,#113170,#113171,#113172,#113173,
#113174,#113175,#113176,#113177,#113178,#113179,#113180,#113181,#113182,
#113183,#113184,#113185,#113186,#113187,#113188,#113189,#113190,#113191,
#113192,#113193,#113194,#113195,#113196,#113197,#113198,#113199,#113200,
#113201,#113202,#113203,#113204,#113205,#113206,#113207,#113208,#113209,
#113210,#113211,#113212,#113213,#113214,#113215,#113216,#113217,#113218,
#113219,#113220,#113221,#113222,#113223,#113224,#113225,#113226,#113227,
#113228,#113229,#113230,#113231,#113232,#113233,#113234,#113235,#113236,
#113237,#113238,#113239,#113240,#113241,#113242,#113243,#113244,#113245,
#113246,#113247,#113248,#113249,#113250,#113251,#113252,#113253,#113254,
#113255,#113256,#113257,#113258),.UNSPECIFIED.,.F.,.F.,(4,2,2,2,2,2,2,2,
2,2,2,2,2,2,2,2,2,2,2,2,2,2,2,2,2,2,2,2,2,2,2,2,2,2,2,2,2,2,2,2,2,2,2,2,
2,2,2,2,2,2,2,2,2,2,2,2,2,2,2,2,2,2,2,2,2,2,2,2,2,2,2,2,2,2,2,2,2,2,2,2,
2,2,2,2,2,2,2,2,2,2,2,2,2,2,2,2,2,2,2,2,2,2,2,2,2,2,2,4),(-2.66731151661852,
-2.64527185279398,-2.59640216442595,-2.58668066625757,-2.58450952792302,
-2.58327612034247,-2.5822027106984,-2.58082465065772,-2.57796472130922,
-2.54188915064359,-2.50916127755015,-2.49278663887684,-2.48599210724353,
-2.48236584360222,-2.47926527249087,-2.47725867411702,-2.47531737148135,
-2.47277568511123,-2.46848045684978,-2.43348606520522,-2.38457210454266,
-2.37475884470456,-2.37257893914507,-2.37134230128741,-2.37026831322801,
-2.36889163335558,-2.36603913620571,-2.32973367110866,-2.27586869803088,
-2.26941107622515,-2.26669839730375,-2.26473602260654,-2.26294429953827,
-2.26008406699031,-2.25322794818502,-2.19978060101934,-2.17412315671989,
-2.16288001130005,-2.16061141503366,-2.15935593733485,-2.15828470191138,
-2.15693621006764,-2.1543104172533,-2.13814252822413,-2.09165928558698,
-2.06369635954698,-2.05735261406887,-2.0546594631257,-2.05270084790813,
-2.05090539161289,-2.04802353856523,-2.04103459607239,-1.9894622732371,
-1.96249380035042,-1.95092069309849,-1.94863343629199,-1.94737395496668,
-1.94630298714801,-1.94495955402626,-1.94235776759311,-1.92677008376512,
-1.92028688316622,-1.9063874221587,-1.87350459214437,-1.85694733158858,
-1.84663922694345,-1.84339073145481,-1.84131737338695,-1.83937653898136,
-1.8368349871214,-1.83253894587197,-1.7973408108906,-1.74809994649225,-1.73871504219033,
-1.73656572820817,-1.73533619628985,-1.734261494231,-1.73287502528677,-1.72997202728907,
-1.69791050362839,-1.66501814149649,-1.6461912354045,-1.63870697009884,
-1.63308477158178,-1.63051922950906,-1.62858160605694,-1.62675311019602,
-1.6242045451054,-1.61752110285484,-1.56212974443479,-1.53778871066859,
-1.52689025439241,-1.52464169684738,-1.52339043512033,-1.5223185437245,
-1.52096378545313,-1.51830969384103,-1.50142768119834,-1.48264098203071,
-1.44967629550916,-1.43302371015258,-1.42267235932078,-1.41941878660761,
-1.41734423982245,-1.41540373324461,-1.41286468844989,-1.40857754252068,
-1.40821110954925),.UNSPECIFIED.);
#1087=B_SPLINE_CURVE_WITH_KNOTS('',3,(#113260,#113261,#113262,#113263,#113264,
#113265,#113266,#113267,#113268,#113269,#113270,#113271,#113272,#113273,
#113274,#113275,#113276,#113277,#113278,#113279,#113280,#113281,#113282,
#113283,#113284,#113285,#113286,#113287,#113288,#113289,#113290,#113291,
#113292,#113293,#113294,#113295,#113296,#113297,#113298,#113299,#113300,
#113301,#113302,#113303,#113304,#113305,#113306,#113307,#113308,#113309,
#113310,#113311,#113312,#113313,#113314,#113315,#113316,#113317,#113318,
#113319,#113320,#113321,#113322,#113323,#113324,#113325,#113326,#113327,
#113328,#113329,#113330,#113331,#113332,#113333,#113334,#113335,#113336,
#113337,#113338,#113339,#113340,#113341,#113342,#113343,#113344,#113345,
#113346,#113347,#113348,#113349,#113350,#113351,#113352,#113353,#113354,
#113355,#113356,#113357,#113358,#113359,#113360,#113361,#113362,#113363,
#113364,#113365,#113366,#113367,#113368,#113369,#113370,#113371,#113372,
#113373,#113374,#113375,#113376,#113377,#113378,#113379,#113380,#113381,
#113382,#113383,#113384,#113385,#113386,#113387,#113388,#113389,#113390,
#113391,#113392,#113393,#113394,#113395,#113396,#113397,#113398,#113399,
#113400,#113401,#113402,#113403,#113404,#113405,#113406,#113407,#113408,
#113409,#113410,#113411,#113412,#113413,#113414,#113415,#113416,#113417,
#113418,#113419,#113420,#113421,#113422,#113423,#113424,#113425,#113426,
#113427,#113428,#113429,#113430,#113431,#113432,#113433,#113434,#113435,
#113436,#113437,#113438,#113439,#113440,#113441,#113442,#113443,#113444,
#113445,#113446,#113447,#113448,#113449,#113450,#113451,#113452,#113453,
#113454,#113455,#113456,#113457,#113458,#113459,#113460,#113461,#113462,
#113463,#113464,#113465,#113466,#113467,#113468,#113469,#113470,#113471,
#113472,#113473,#113474,#113475,#113476,#113477,#113478,#113479,#113480,
#113481),.UNSPECIFIED.,.F.,.F.,(4,2,2,2,2,2,2,2,2,2,2,2,2,2,2,2,2,2,2,2,
2,2,2,2,2,2,2,2,2,2,2,2,2,2,2,2,2,2,2,2,2,2,2,2,2,2,2,2,2,2,2,2,2,2,2,2,
2,2,2,2,2,2,2,2,2,2,2,2,2,2,2,2,2,2,2,2,2,2,2,2,2,2,2,2,2,2,2,2,2,2,2,2,
2,2,2,2,2,2,2,2,2,2,2,2,2,2,2,2,2,2,4),(-1.25960928830829,-1.2101117100023,
-1.20367844137046,-1.20117008054523,-1.199352222804,-1.19740893200012,-1.19480672582928,
-1.18898300427882,-1.1651496649384,-1.11614970833641,-1.09779132516482,
-1.09505198479947,-1.09369779538215,-1.09262569429207,-1.091373276574,-1.08912117655308,
-1.07817666520136,-1.05366048074937,-0.998557406439847,-0.991850207608283,
-0.989297591648701,-0.987467723994383,-0.985530047576476,-0.982966790367328,
-0.977359055330417,-0.929075722515686,-0.888723725139279,-0.88401133694563,
-0.882271358220582,-0.881246072913938,-0.8801546388005,-0.878645349061097,
-0.875062851212622,-0.870037768440905,-0.856214069864457,-0.833861217404663,
-0.787184926908894,-0.779989388727153,-0.777074382950992,-0.77527386731896,
-0.773322046068984,-0.770660414921931,-0.764492394996883,-0.737950131824738,
-0.698622662555807,-0.687289036438417,-0.673503748242721,-0.671211291792618,
-0.669826541041902,-0.668750089367687,-0.66753497130969,-0.665449688919358,
-0.656908818831688,-0.640350240953428,-0.598278838009361,-0.571099362543136,
-0.566971819389208,-0.564478990064701,-0.562545247774404,-0.560449585972271,
-0.557102081837438,-0.545904454396437,-0.527329496232905,-0.484798680915965,
-0.462028237451359,-0.459170516350986,-0.457791888052064,-0.456715623980624,
-0.45547461932324,-0.453286919802481,-0.443433527039587,-0.394232083469812,
-0.359839378033064,-0.355551683815739,-0.35300968797315,-0.351065311500599,
-0.348985015352746,-0.34571896466666,-0.335297135909555,-0.31850522127589,
-0.258883319425073,-0.24929424390937,-0.247244906115271,-0.245918287774539,
-0.244851249483811,-0.243841532970202,-0.241869149982625,-0.234451219181236,
-0.220918010117147,-0.192337919011177,-0.147271566506105,-0.143024761003124,
-0.140506700568832,-0.138580701068639,-0.136520268764679,-0.133286118483809,
-0.122977204712598,-0.106384720379404,-0.084518600633027,-0.0739382468765593,
-0.0616383509458848,-0.0559548978942787,-0.0377854527850606,-0.0350634000144293,
-0.0337175099674206,-0.0326484304901323,-0.0316335621886587,-0.0303960653396582,
-0.0285520766491967,-0.0215326330435678,-0.000655563710816865),
 .UNSPECIFIED.);
#1088=B_SPLINE_CURVE_WITH_KNOTS('',3,(#113482,#113483,#113484,#113485,#113486,
#113487,#113488,#113489,#113490,#113491,#113492,#113493,#113494),
 .UNSPECIFIED.,.F.,.F.,(4,3,3,3,4),(-3.84103903298818,-3.73916989476587,
-3.63740763932563,-3.5357185998273,-3.49054210138362),.UNSPECIFIED.);
#1089=B_SPLINE_CURVE_WITH_KNOTS('',3,(#113497,#113498,#113499,#113500,#113501,
#113502,#113503,#113504,#113505,#113506,#113507,#113508,#113509,#113510,
#113511,#113512,#113513,#113514,#113515,#113516,#113517,#113518,#113519,
#113520,#113521,#113522,#113523,#113524,#113525,#113526,#113527,#113528,
#113529,#113530,#113531,#113532,#113533,#113534,#113535,#113536,#113537,
#113538,#113539,#113540,#113541,#113542,#113543,#113544,#113545,#113546,
#113547,#113548,#113549,#113550,#113551,#113552,#113553,#113554,#113555,
#113556,#113557,#113558,#113559,#113560,#113561,#113562,#113563,#113564,
#113565,#113566,#113567,#113568,#113569,#113570,#113571,#113572,#113573,
#113574,#113575,#113576,#113577,#113578,#113579,#113580,#113581,#113582,
#113583,#113584,#113585,#113586,#113587,#113588,#113589,#113590,#113591,
#113592,#113593,#113594,#113595,#113596,#113597,#113598,#113599,#113600,
#113601,#113602,#113603,#113604,#113605,#113606,#113607,#113608,#113609,
#113610,#113611,#113612,#113613,#113614,#113615,#113616,#113617,#113618,
#113619,#113620,#113621,#113622,#113623,#113624,#113625,#113626,#113627,
#113628,#113629,#113630,#113631,#113632,#113633,#113634,#113635,#113636,
#113637,#113638,#113639,#113640,#113641,#113642,#113643,#113644,#113645,
#113646,#113647,#113648,#113649,#113650,#113651,#113652,#113653,#113654,
#113655,#113656,#113657,#113658,#113659,#113660,#113661,#113662,#113663,
#113664,#113665,#113666,#113667,#113668,#113669,#113670,#113671,#113672,
#113673,#113674,#113675,#113676,#113677,#113678,#113679,#113680,#113681,
#113682,#113683,#113684,#113685,#113686,#113687,#113688,#113689,#113690,
#113691,#113692,#113693,#113694,#113695,#113696,#113697,#113698,#113699,
#113700,#113701,#113702,#113703,#113704,#113705,#113706,#113707),
 .UNSPECIFIED.,.F.,.F.,(4,3,3,3,3,3,3,3,3,3,3,3,3,3,3,3,3,3,3,3,3,3,3,3,
3,3,3,3,3,3,3,3,3,3,3,3,3,3,3,3,3,3,3,3,3,3,3,3,3,3,3,3,3,3,3,3,3,3,3,3,
3,3,3,3,3,3,3,3,3,3,4),(7.94826257357117,8.03933917600296,8.13040880367845,
8.22150057347938,8.28490746193705,8.37600652726715,8.46708731777336,8.55817079881158,
8.64924995373853,8.74034821484711,8.77225495969805,8.86358513560277,8.9548986330717,
9.04621476194116,9.1375258664909,9.22885308111593,9.25960245745905,9.35004385837792,
9.44046482582385,9.53089150074111,9.62131715354628,9.7117720080883,9.74694995522006,
9.83977478998513,9.93258815792015,10.025393459506,10.1181816912061,10.2109546401573,
10.2342974529811,10.3226295283866,10.410939313145,10.4992670123095,10.5876031247876,
10.6759967918602,10.7216449507421,10.8173001765085,10.9152232445072,11.0108032234786,
11.1098978359908,11.2089924485031,11.2974448715171,11.3858946564481,11.4743908456245,
11.562911632656,11.6515132694445,11.6963399462641,11.7845989400825,11.872784715549,
11.9609169884106,12.0496817325825,12.1377840060822,12.22589474066,12.31403174787,
12.403282546349,12.4915728517076,12.5813038967469,12.6710349417861,12.7563671078331,
12.8415835245525,12.9267079378408,13.011763973049,13.0967844578901,13.1817894416759,
13.2668001713248,13.3518378971159,13.4369760189292,13.5221713946028,13.6075027101629,
13.6457299373081,13.775760012771,13.8747245557601),.UNSPECIFIED.);
#1090=B_SPLINE_CURVE_WITH_KNOTS('',3,(#113708,#113709,#113710,#113711,#113712,
#113713,#113714,#113715,#113716,#113717,#113718,#113719,#113720,#113721,
#113722,#113723),.UNSPECIFIED.,.F.,.F.,(4,3,3,3,3,4),(13.8747245559395,
13.9640191448913,14.0502852614935,14.1364993985763,14.2226809109192,14.2319029117468),
 .UNSPECIFIED.);
#1091=B_SPLINE_CURVE_WITH_KNOTS('',3,(#113725,#113726,#113727,#113728,#113729,
#113730,#113731,#113732,#113733,#113734,#113735,#113736,#113737),
 .UNSPECIFIED.,.F.,.F.,(4,3,3,3,4),(-10.49477808198,-10.4064650448213,-10.3181276030325,
-10.2342974529811,-10.1382057107015),.UNSPECIFIED.);
#1092=B_SPLINE_CURVE_WITH_KNOTS('',3,(#113738,#113739,#113740,#113741,#113742,
#113743,#113744,#113745,#113746,#113747,#113748,#113749,#113750,#113751,
#113752,#113753,#113754,#113755,#113756,#113757,#113758,#113759,#113760,
#113761,#113762,#113763,#113764,#113765,#113766,#113767,#113768,#113769,
#113770,#113771,#113772,#113773,#113774,#113775,#113776,#113777,#113778,
#113779,#113780,#113781,#113782,#113783,#113784,#113785,#113786,#113787,
#113788,#113789),.UNSPECIFIED.,.F.,.F.,(4,2,2,2,2,2,2,2,2,2,2,2,2,2,2,2,
2,2,2,2,2,2,2,2,2,4),(1.80129261558726,1.89085724581047,1.95815067052896,
2.04087191045445,2.16781420139301,2.30159864887717,2.38018379042639,2.50753373614498,
2.58026236347961,2.72352021082451,2.80830108353013,2.89228193268548,3.05888345033062,
3.13851550682636,3.22568042995156,3.3096718361238,3.47401737896509,3.55360256241736,
3.69279581467806,3.77292072282912,3.8403007617186,3.92420528255271,4.09335994867267,
4.20858348747028,4.27205568576047,4.33574044619876),.UNSPECIFIED.);
#1093=B_SPLINE_CURVE_WITH_KNOTS('',3,(#113791,#113792,#113793,#113794,#113795,
#113796,#113797,#113798,#113799,#113800,#113801,#113802,#113803,#113804,
#113805,#113806,#113807,#113808,#113809,#113810,#113811,#113812,#113813,
#113814,#113815,#113816,#113817,#113818,#113819,#113820,#113821,#113822,
#113823,#113824,#113825,#113826,#113827,#113828,#113829,#113830,#113831,
#113832,#113833,#113834,#113835,#113836,#113837,#113838,#113839,#113840,
#113841,#113842,#113843,#113844),.UNSPECIFIED.,.F.,.F.,(4,2,2,2,2,2,2,2,
2,2,2,2,2,2,2,2,2,2,2,2,2,2,2,2,2,2,4),(-2.84070125419267,-2.78020516982207,
-2.65435179246817,-2.57659131794918,-2.4969909063458,-2.32946562003716,
-2.24549752924312,-2.17252648783871,-2.05532984848559,-1.97398064924123,
-1.85252487658554,-1.68460873253962,-1.51626211229805,-1.442685683892,-1.30223160143275,
-1.22322244978935,-1.10078998236665,-1.03027786474523,-0.859932808523249,
-0.777908083368037,-0.656316970603006,-0.575106553635839,-0.460076680830133,
-0.393722373564878,-0.309798675310045,-0.154355410284551,-0.153225104208862),
 .UNSPECIFIED.);
#1094=B_SPLINE_CURVE_WITH_KNOTS('',3,(#113846,#113847,#113848,#113849,#113850,
#113851,#113852,#113853,#113854,#113855,#113856,#113857,#113858,#113859,
#113860,#113861,#113862,#113863,#113864,#113865,#113866,#113867,#113868,
#113869,#113870,#113871,#113872,#113873,#113874,#113875,#113876,#113877,
#113878,#113879,#113880,#113881,#113882,#113883,#113884,#113885,#113886,
#113887,#113888,#113889,#113890,#113891,#113892,#113893,#113894,#113895,
#113896,#113897,#113898,#113899,#113900,#113901,#113902,#113903,#113904,
#113905,#113906,#113907,#113908,#113909,#113910,#113911,#113912,#113913,
#113914,#113915,#113916,#113917,#113918,#113919,#113920,#113921,#113922,
#113923,#113924,#113925,#113926,#113927,#113928,#113929,#113930,#113931,
#113932,#113933,#113934,#113935,#113936,#113937,#113938,#113939,#113940,
#113941,#113942,#113943,#113944,#113945,#113946,#113947,#113948,#113949,
#113950,#113951,#113952,#113953,#113954,#113955,#113956,#113957,#113958,
#113959,#113960,#113961,#113962,#113963,#113964,#113965,#113966,#113967,
#113968,#113969,#113970,#113971,#113972,#113973,#113974,#113975,#113976,
#113977,#113978,#113979,#113980,#113981,#113982,#113983,#113984,#113985,
#113986,#113987,#113988,#113989,#113990,#113991,#113992,#113993,#113994,
#113995,#113996,#113997,#113998,#113999,#114000,#114001,#114002,#114003,
#114004,#114005,#114006,#114007,#114008,#114009,#114010,#114011,#114012,
#114013,#114014,#114015,#114016,#114017,#114018,#114019,#114020,#114021,
#114022,#114023,#114024,#114025,#114026,#114027,#114028,#114029,#114030,
#114031,#114032,#114033,#114034,#114035,#114036,#114037,#114038,#114039,
#114040,#114041,#114042,#114043,#114044,#114045,#114046,#114047,#114048,
#114049,#114050,#114051,#114052,#114053,#114054,#114055,#114056,#114057,
#114058,#114059),.UNSPECIFIED.,.F.,.F.,(4,3,3,3,3,3,3,3,3,3,3,3,3,3,3,3,
3,3,3,3,3,3,3,3,3,3,3,3,3,3,3,3,3,3,3,3,3,3,3,3,3,3,3,3,3,3,3,3,3,3,3,3,
3,3,3,3,3,3,3,3,3,3,3,3,3,3,3,3,3,3,3,4),(20.5146317045532,20.6057411498849,
20.6968511934372,20.7879526845016,20.879076798166,20.9559424037231,21.0470612888528,
21.1381622720158,21.2292662857086,21.3203661134592,21.4114850765015,21.4432899014841,
21.5344090066244,21.6255102040649,21.7166144214506,21.8077144461872,21.8988335947371,
21.9306373992451,22.0217552957911,22.1128552867068,22.2039583127407,22.2950571581876,
22.3861751549738,22.4179848970061,22.5091059022033,22.6002090058036,22.6913151191521,
22.7824170287616,22.8735380301917,22.9053323947671,22.9964483174135,23.0875463337701,
23.1786474040368,23.2697443099321,23.3608604070626,23.3926798925281,23.4838001385027,
23.5749024646883,23.6660077819953,23.7571088869989,23.8482290782052,23.8800273902891,
23.9711543330786,24.0622634337937,24.1533755706366,24.2444835024034,24.3356104731702,
24.3673748880501,24.4584575658978,24.5495221768875,24.6405899421199,24.7316536918334,
24.82273712851,24.8547223858111,24.9459385829945,25.037137248471,25.1283384958124,
25.2195350261609,25.3107491009262,25.3420698835722,25.4329784991865,25.5238689926783,
25.6147642806767,25.7056569563173,25.7965727963716,25.8294173813332,25.9210352148413,
26.0126339675887,26.1042287090123,26.1958136721735,26.2874053890112,26.3167648790942),
 .UNSPECIFIED.);
#1095=B_SPLINE_CURVE_WITH_KNOTS('',3,(#114063,#114064,#114065,#114066,#114067,
#114068,#114069,#114070),.UNSPECIFIED.,.F.,.F.,(4,1,1,1,1,4),(17.9342415705864,
18.8587793842596,19.8576158342214,20.8564522841833,21.8552887341452,21.9911485751286),
 .UNSPECIFIED.);
#1096=B_SPLINE_CURVE_WITH_KNOTS('',3,(#114071,#114072,#114073,#114074,#114075,
#114076),.UNSPECIFIED.,.F.,.F.,(4,1,1,4),(21.9911485751286,22.854125184107,
23.8529616340689,24.2176478004184),.UNSPECIFIED.);
#1097=B_SPLINE_CURVE_WITH_KNOTS('',3,(#114078,#114079,#114080,#114081,#114082,
#114083,#114084,#114085,#114086,#114087,#114088,#114089,#114090,#114091,
#114092,#114093,#114094,#114095,#114096,#114097,#114098,#114099,#114100,
#114101,#114102,#114103,#114104,#114105,#114106,#114107,#114108,#114109,
#114110,#114111,#114112,#114113,#114114,#114115,#114116,#114117,#114118,
#114119,#114120,#114121,#114122,#114123,#114124,#114125,#114126,#114127,
#114128,#114129,#114130,#114131,#114132,#114133,#114134,#114135,#114136,
#114137,#114138,#114139,#114140,#114141,#114142,#114143,#114144,#114145,
#114146,#114147),.UNSPECIFIED.,.F.,.F.,(4,3,3,3,3,3,3,3,3,3,3,3,3,3,3,3,
3,3,3,3,3,3,3,4),(21.9911487995909,22.0999040367044,22.2090425458686,22.3187160667875,
22.3893184515875,22.487921335874,22.5863839114419,22.6866052852054,22.7848896824335,
22.883141107753,22.9813890373117,23.0830805033711,23.1814697140479,23.2848123077986,
23.3881549015493,23.4916866771327,23.5901227234309,23.6884632070921,23.7867377206608,
23.8849757858551,23.9832411509404,24.0815224781616,24.1798939405651,24.2164091062169),
 .UNSPECIFIED.);
#1098=B_SPLINE_CURVE_WITH_KNOTS('',3,(#114148,#114149,#114150,#114151,#114152,
#114153,#114154,#114155),.UNSPECIFIED.,.F.,.F.,(4,1,1,1,1,4),(17.9335273147171,
18.39397265174,19.3928091017018,20.3916455516637,21.3904820016256,21.9911485751286),
 .UNSPECIFIED.);
#1099=B_SPLINE_CURVE_WITH_KNOTS('',3,(#114158,#114159,#114160,#114161,#114162,
#114163,#114164,#114165),.UNSPECIFIED.,.F.,.F.,(4,1,1,1,1,4),(17.9342415897067,
18.8587793842596,19.8576158342214,20.8564522841833,21.8552887341452,21.9911485751286),
 .UNSPECIFIED.);
#1100=B_SPLINE_CURVE_WITH_KNOTS('',3,(#114166,#114167,#114168,#114169,#114170,
#114171),.UNSPECIFIED.,.F.,.F.,(4,1,1,4),(21.9911485751286,22.854125184107,
23.8529616340689,24.2176478214031),.UNSPECIFIED.);
#1101=B_SPLINE_CURVE_WITH_KNOTS('',3,(#114173,#114174,#114175,#114176,#114177,
#114178,#114179,#114180,#114181,#114182,#114183,#114184,#114185,#114186,
#114187,#114188,#114189,#114190,#114191,#114192,#114193,#114194,#114195,
#114196,#114197,#114198,#114199,#114200,#114201,#114202,#114203,#114204,
#114205,#114206,#114207,#114208,#114209,#114210,#114211,#114212,#114213,
#114214,#114215,#114216,#114217,#114218,#114219,#114220,#114221,#114222,
#114223,#114224,#114225,#114226,#114227,#114228,#114229,#114230,#114231,
#114232,#114233,#114234,#114235,#114236,#114237,#114238,#114239,#114240,
#114241,#114242),.UNSPECIFIED.,.F.,.F.,(4,3,3,3,3,3,3,3,3,3,3,3,3,3,3,3,
3,3,3,3,3,3,3,4),(21.9911487995816,22.0999040743052,22.2090426220591,22.3187161819304,
22.3893184515875,22.487921325434,22.5863838904609,22.6866052668469,22.7848896533628,
22.8831410679294,22.9813889867089,23.083080465419,23.1814696653607,23.284812283455,
23.3881549015493,23.4916866796568,23.5901227238994,23.6884632054536,23.7867377168667,
23.8849757798596,23.983241142689,24.081522467619,24.1798939277032,24.2164091264089),
 .UNSPECIFIED.);
#1102=B_SPLINE_CURVE_WITH_KNOTS('',3,(#114243,#114244,#114245,#114246,#114247,
#114248,#114249,#114250),.UNSPECIFIED.,.F.,.F.,(4,1,1,1,1,4),(17.9335273553052,
18.39397265174,19.3928091017018,20.3916455516637,21.3904820016256,21.9911485751286),
 .UNSPECIFIED.);
#1103=B_SPLINE_CURVE_WITH_KNOTS('',3,(#114253,#114254,#114255,#114256,#114257,
#114258,#114259,#114260),.UNSPECIFIED.,.F.,.F.,(4,1,1,1,1,4),(17.9342415884722,
18.8587793842595,19.8576158342214,20.8564522841833,21.8552887341452,21.9911485751286),
 .UNSPECIFIED.);
#1104=B_SPLINE_CURVE_WITH_KNOTS('',3,(#114261,#114262,#114263,#114264,#114265,
#114266),.UNSPECIFIED.,.F.,.F.,(4,1,1,4),(21.9911485751286,22.854125184107,
23.8529616340689,24.2176478200484),.UNSPECIFIED.);
#1105=B_SPLINE_CURVE_WITH_KNOTS('',3,(#114268,#114269,#114270,#114271,#114272,
#114273,#114274,#114275,#114276,#114277,#114278,#114279,#114280,#114281,
#114282,#114283,#114284,#114285,#114286,#114287,#114288,#114289,#114290,
#114291,#114292,#114293,#114294,#114295,#114296,#114297,#114298,#114299,
#114300,#114301,#114302,#114303,#114304,#114305,#114306,#114307,#114308,
#114309,#114310,#114311,#114312,#114313,#114314,#114315,#114316,#114317,
#114318,#114319,#114320,#114321,#114322,#114323,#114324,#114325,#114326,
#114327,#114328,#114329,#114330,#114331,#114332,#114333,#114334,#114335,
#114336,#114337),.UNSPECIFIED.,.F.,.F.,(4,3,3,3,3,3,3,3,3,3,3,3,3,3,3,3,
3,3,3,3,3,3,3,4),(21.9911487995803,22.0999040794723,22.2090426325292,22.3187161977535,
22.3893184515875,22.4879213239996,22.5863838875782,22.6866052643246,22.7848896493685,
22.8831410624578,22.9813889797561,23.0830804602044,23.1814696586711,23.2848122801102,
23.3881549015493,23.4916866794652,23.5901227234261,23.6884632046911,23.7867377158082,
23.8849757784984,23.9832411410165,24.0815224656302,24.179893925392,24.2164091248765),
 .UNSPECIFIED.);
#1106=B_SPLINE_CURVE_WITH_KNOTS('',3,(#114338,#114339,#114340,#114341,#114342,
#114343,#114344,#114345),.UNSPECIFIED.,.F.,.F.,(4,1,1,1,1,4),(17.9335273566036,
18.39397265174,19.3928091017018,20.3916455516637,21.3904820016256,21.9911485751286),
 .UNSPECIFIED.);
#1107=B_SPLINE_CURVE_WITH_KNOTS('',3,(#114348,#114349,#114350,#114351,#114352,
#114353,#114354,#114355),.UNSPECIFIED.,.F.,.F.,(4,1,1,1,1,4),(17.9342415312022,
18.8587793842595,19.8576158342214,20.8564522841833,21.8552887341452,21.9911485751286),
 .UNSPECIFIED.);
#1108=B_SPLINE_CURVE_WITH_KNOTS('',3,(#114356,#114357,#114358,#114359,#114360,
#114361),.UNSPECIFIED.,.F.,.F.,(4,1,1,4),(21.9911485751286,22.854125184107,
23.8529616340689,24.2176477571914),.UNSPECIFIED.);
#1109=B_SPLINE_CURVE_WITH_KNOTS('',3,(#114363,#114364,#114365,#114366,#114367,
#114368,#114369,#114370,#114371,#114372,#114373,#114374,#114375,#114376,
#114377,#114378,#114379,#114380,#114381,#114382,#114383,#114384,#114385,
#114386,#114387,#114388,#114389,#114390,#114391,#114392,#114393,#114394,
#114395,#114396,#114397,#114398,#114399,#114400,#114401,#114402,#114403,
#114404,#114405,#114406,#114407,#114408,#114409,#114410,#114411,#114412,
#114413,#114414,#114415,#114416,#114417,#114418,#114419,#114420,#114421,
#114422,#114423,#114424,#114425,#114426,#114427,#114428,#114429,#114430,
#114431,#114432),.UNSPECIFIED.,.F.,.F.,(4,3,3,3,3,3,3,3,3,3,3,3,3,3,3,3,
3,3,3,3,3,3,3,4),(21.9911487995834,22.0999040669592,22.2090426071739,22.318716159435,
22.3893184515875,22.4879213274736,22.5863838945597,22.6866052704334,22.7848896590419,
22.8831410757092,22.9813889965944,23.0830804728331,23.181469674872,23.2848122882107,
23.3881549015493,23.4916866715276,23.5901227161827,23.6884631981554,23.7867377099928,
23.884975773415,23.9832411366681,24.081522462026,24.1798939225121,24.2164090613759),
 .UNSPECIFIED.);
#1110=B_SPLINE_CURVE_WITH_KNOTS('',3,(#114433,#114434,#114435,#114436,#114437,
#114438,#114439,#114440),.UNSPECIFIED.,.F.,.F.,(4,1,1,1,1,4),(17.9335272866486,
18.39397265174,19.3928091017018,20.3916455516637,21.3904820016256,21.9911485751286),
 .UNSPECIFIED.);
#1111=B_SPLINE_CURVE_WITH_KNOTS('',3,(#114443,#114444,#114445,#114446,#114447,
#114448,#114449,#114450,#114451,#114452,#114453,#114454),.UNSPECIFIED.,
 .F.,.F.,(4,1,1,1,1,1,1,1,1,4),(17.9329414843961,18.1884603353201,18.6758078330811,
19.1631553308421,19.6505028286031,20.1378503263641,20.6251978241251,21.1125453218861,
21.5998928196471,21.991148557883),.UNSPECIFIED.);
#1112=B_SPLINE_CURVE_WITH_KNOTS('',3,(#114455,#114456,#114457,#114458,#114459,
#114460,#114461,#114462,#114463,#114464,#114465,#114466,#114467,#114468,
#114469,#114470,#114471,#114472,#114473,#114474,#114475,#114476,#114477,
#114478,#114479,#114480,#114481,#114482,#114483,#114484,#114485,#114486,
#114487,#114488,#114489,#114490,#114491,#114492,#114493,#114494,#114495,
#114496,#114497,#114498,#114499,#114500,#114501,#114502,#114503,#114504,
#114505,#114506,#114507,#114508,#114509,#114510,#114511,#114512,#114513,
#114514,#114515,#114516,#114517,#114518,#114519,#114520,#114521,#114522,
#114523,#114524,#114525,#114526,#114527,#114528,#114529,#114530,#114531,
#114532,#114533,#114534,#114535,#114536),.UNSPECIFIED.,.F.,.F.,(4,3,3,3,
3,3,3,3,3,3,3,3,3,3,3,3,3,3,3,3,3,3,3,3,3,3,3,4),(21.9911485751285,22.0872403174081,
22.1717077643695,22.2561544844513,22.3406177643316,22.4250871456575,22.5096125640496,
22.5745878151691,22.6660514455681,22.7575040081467,22.8489019715955,22.9402390467649,
23.0314631630385,23.0619353129301,23.1465167513392,23.2310954406081,23.3157173860693,
23.4003602647289,23.4850816883211,23.5492828106911,23.633669288197,23.7179929955514,
23.8022695765466,23.8865146391538,23.970761703403,24.0550059922274,24.139296875598,
24.2156473321997),.UNSPECIFIED.);
#1113=B_SPLINE_CURVE_WITH_KNOTS('',3,(#114538,#114539,#114540,#114541,#114542,
#114543,#114544,#114545,#114546,#114547,#114548,#114549,#114550,#114551,
#114552,#114553,#114554,#114555,#114556,#114557,#114558,#114559,#114560,
#114561,#114562,#114563,#114564,#114565,#114566,#114567,#114568,#114569,
#114570,#114571,#114572,#114573,#114574,#114575,#114576,#114577,#114578,
#114579,#114580,#114581,#114582,#114583,#114584,#114585,#114586,#114587,
#114588,#114589,#114590,#114591,#114592,#114593,#114594,#114595,#114596,
#114597,#114598,#114599,#114600,#114601,#114602,#114603,#114604,#114605,
#114606,#114607,#114608,#114609,#114610,#114611,#114612,#114613,#114614,
#114615,#114616,#114617,#114618,#114619,#114620,#114621,#114622),
 .UNSPECIFIED.,.F.,.F.,(4,3,3,3,3,3,3,3,3,3,3,3,3,3,3,3,3,3,3,3,3,3,3,3,
3,3,3,3,4),(21.9911485753162,22.0800609495919,22.168999417996,22.1971692907241,
22.2842691742849,22.3713525460866,22.4584393273926,22.5455216572055,22.6326240181457,
22.6845167884851,22.7716275763734,22.8587214790213,22.9458181342347,23.0329099438452,
23.120021097721,23.1718642862461,23.2591953323291,23.3465109695105,23.4338293669418,
23.5211423678883,23.60847190326,23.6592117840071,23.7456953098164,23.832159927636,
23.9186299638456,24.005097953844,24.0915948443439,24.1465592817681,24.2161266164728),
 .UNSPECIFIED.);
#1114=B_SPLINE_CURVE_WITH_KNOTS('',3,(#114623,#114624,#114625,#114626,#114627,
#114628,#114629,#114630,#114631,#114632,#114633,#114634,#114635,#114636,
#114637,#114638,#114639,#114640,#114641,#114642,#114643,#114644,#114645,
#114646,#114647,#114648,#114649,#114650,#114651,#114652,#114653,#114654,
#114655,#114656,#114657,#114658,#114659,#114660,#114661,#114662,#114663,
#114664,#114665,#114666,#114667,#114668,#114669,#114670,#114671,#114672,
#114673,#114674,#114675,#114676,#114677,#114678,#114679,#114680,#114681,
#114682,#114683,#114684,#114685,#114686,#114687,#114688,#114689,#114690,
#114691,#114692,#114693,#114694,#114695,#114696,#114697,#114698,#114699,
#114700,#114701,#114702,#114703,#114704,#114705,#114706,#114707,#114708,
#114709,#114710,#114711,#114712,#114713,#114714,#114715,#114716,#114717,
#114718,#114719,#114720,#114721,#114722,#114723,#114724,#114725,#114726,
#114727,#114728,#114729,#114730,#114731,#114732,#114733,#114734,#114735,
#114736,#114737,#114738,#114739,#114740,#114741,#114742,#114743,#114744,
#114745,#114746,#114747,#114748,#114749,#114750,#114751,#114752,#114753,
#114754,#114755,#114756,#114757,#114758,#114759,#114760,#114761,#114762,
#114763,#114764,#114765,#114766,#114767,#114768,#114769,#114770,#114771,
#114772,#114773,#114774,#114775,#114776),.UNSPECIFIED.,.F.,.F.,(4,3,3,3,
3,3,3,3,3,3,3,3,3,3,3,3,3,3,3,3,3,3,3,3,3,3,3,3,3,3,3,3,3,3,3,3,3,3,3,3,
3,3,3,3,3,3,3,3,3,3,3,4),(17.9329528346437,18.0243119531418,18.1114270891671,
18.1985409744401,18.2856718326635,18.298389308636,18.3855180493059,18.4726302285909,
18.559745465589,18.6468559845724,18.7339858790278,18.785736806397,18.8728666485425,
18.959979950145,19.0470963297829,19.1342080001734,19.2213390494988,19.273084304158,
19.3602139689286,19.4473270846037,19.534443267337,19.6215547350878,19.7086855747234,
19.760431801919,19.8475621199502,19.9346758967653,20.0217927459667,20.1089048815892,
20.1960363853822,20.24777929968,20.3349058916832,20.4220159234169,20.5091290354302,
20.5962374473094,20.6833652806739,20.735126797441,20.8222649721476,20.9093866302891,
20.9965113211569,21.0836312571589,21.1707704295162,21.222474295202,21.3095858862927,
21.3966808826214,21.4837790530665,21.5708726121089,21.6579858588927,21.709821792963,
21.797454164746,21.8850673211435,21.9726698643262,21.9911485751285),
 .UNSPECIFIED.);
#1115=B_SPLINE_CURVE_WITH_KNOTS('',3,(#114779,#114780,#114781,#114782,#114783,
#114784,#114785,#114786,#114787,#114788,#114789,#114790),.UNSPECIFIED.,
 .F.,.F.,(4,1,1,1,1,1,1,1,1,4),(17.9329414836179,18.1884603353201,18.6758078330811,
19.1631553308421,19.6505028286031,20.1378503263641,20.6251978241251,21.1125453218861,
21.5998928196471,21.9911485578925),.UNSPECIFIED.);
#1116=B_SPLINE_CURVE_WITH_KNOTS('',3,(#114791,#114792,#114793,#114794,#114795,
#114796,#114797,#114798,#114799,#114800,#114801,#114802,#114803,#114804,
#114805,#114806,#114807,#114808,#114809,#114810,#114811,#114812,#114813,
#114814,#114815,#114816,#114817,#114818,#114819,#114820,#114821,#114822,
#114823,#114824,#114825,#114826,#114827,#114828,#114829,#114830,#114831,
#114832,#114833,#114834,#114835,#114836,#114837,#114838,#114839,#114840,
#114841,#114842,#114843,#114844,#114845,#114846,#114847,#114848,#114849,
#114850,#114851,#114852,#114853,#114854,#114855,#114856,#114857,#114858,
#114859,#114860,#114861,#114862,#114863,#114864,#114865,#114866,#114867,
#114868,#114869,#114870,#114871,#114872),.UNSPECIFIED.,.F.,.F.,(4,3,3,3,
3,3,3,3,3,3,3,3,3,3,3,3,3,3,3,3,3,3,3,3,3,3,3,4),(21.9911485751285,22.0872403174081,
22.1717043008718,22.256147550065,22.3406073668107,22.425073290183,22.5095952809818,
22.5745878151691,22.6660564577372,22.7575140633748,22.8489170049659,22.9402589752051,
23.0314877939314,23.0619353129301,23.1465147382964,23.2310914061767,23.3157113292587,
23.4003521854755,23.4850716002667,23.5492828106911,23.6336693594472,23.7179931343229,
23.8022697790428,23.8865149015084,23.9707620193541,24.0550063583272,24.1392972858986,
24.2156474862923),.UNSPECIFIED.);
#1117=B_SPLINE_CURVE_WITH_KNOTS('',3,(#114874,#114875,#114876,#114877,#114878,
#114879,#114880,#114881,#114882,#114883,#114884,#114885,#114886,#114887,
#114888,#114889,#114890,#114891,#114892,#114893,#114894,#114895,#114896,
#114897,#114898,#114899,#114900,#114901,#114902,#114903,#114904,#114905,
#114906,#114907,#114908,#114909,#114910,#114911,#114912,#114913,#114914,
#114915,#114916,#114917,#114918,#114919,#114920,#114921,#114922,#114923,
#114924,#114925,#114926,#114927,#114928,#114929,#114930,#114931,#114932,
#114933,#114934,#114935,#114936,#114937,#114938,#114939,#114940,#114941,
#114942,#114943,#114944,#114945,#114946,#114947,#114948,#114949,#114950,
#114951,#114952,#114953,#114954,#114955,#114956,#114957,#114958),
 .UNSPECIFIED.,.F.,.F.,(4,3,3,3,3,3,3,3,3,3,3,3,3,3,3,3,3,3,3,3,3,3,3,3,
3,3,3,3,4),(21.9911485753162,22.0800610136685,22.1689995435299,22.1971692907241,
22.2842690753762,22.3713523483423,22.4584390318698,22.5455212647318,22.6326235308353,
22.6845167884851,22.7716274880237,22.8587213011356,22.9458178659101,23.0329095847879,
23.1200206482753,23.1718642862461,23.2591959782146,23.3465122652369,23.4338313118415,
23.5211449598873,23.6084751333609,23.6592117840071,23.745693612034,23.8321565252023,
23.9186248608383,24.0050911555493,24.0915863725887,24.1465592817681,24.2161265625725),
 .UNSPECIFIED.);
#1118=B_SPLINE_CURVE_WITH_KNOTS('',3,(#114959,#114960,#114961,#114962,#114963,
#114964,#114965,#114966,#114967,#114968,#114969,#114970,#114971,#114972,
#114973,#114974,#114975,#114976,#114977,#114978,#114979,#114980,#114981,
#114982,#114983,#114984,#114985,#114986,#114987,#114988,#114989,#114990,
#114991,#114992,#114993,#114994,#114995,#114996,#114997,#114998,#114999,
#115000,#115001,#115002,#115003,#115004,#115005,#115006,#115007,#115008,
#115009,#115010,#115011,#115012,#115013,#115014,#115015,#115016,#115017,
#115018,#115019,#115020,#115021,#115022,#115023,#115024,#115025,#115026,
#115027,#115028,#115029,#115030,#115031,#115032,#115033,#115034,#115035,
#115036,#115037,#115038,#115039,#115040,#115041,#115042,#115043,#115044,
#115045,#115046,#115047,#115048,#115049,#115050,#115051,#115052,#115053,
#115054,#115055,#115056,#115057,#115058,#115059,#115060,#115061,#115062,
#115063,#115064,#115065,#115066,#115067,#115068,#115069,#115070,#115071,
#115072,#115073,#115074,#115075,#115076,#115077,#115078,#115079,#115080,
#115081,#115082,#115083,#115084,#115085,#115086,#115087,#115088,#115089,
#115090,#115091,#115092,#115093,#115094,#115095,#115096,#115097,#115098,
#115099,#115100,#115101,#115102,#115103,#115104,#115105,#115106,#115107,
#115108,#115109,#115110,#115111,#115112),.UNSPECIFIED.,.F.,.F.,(4,3,3,3,
3,3,3,3,3,3,3,3,3,3,3,3,3,3,3,3,3,3,3,3,3,3,3,3,3,3,3,3,3,3,3,3,3,3,3,3,
3,3,3,3,3,3,3,3,3,3,3,4),(17.932952833811,18.0243119525172,18.1114270941441,
18.1985409850432,18.2856718488903,18.298389308636,18.3855180458292,18.4726302215735,
18.5597454549696,18.6468559703248,18.7339858611432,18.785736806397,18.8728666494913,
18.9599799520757,19.0470963327356,19.1342080041683,19.2213390545579,19.273084304158,
19.3602139685927,19.4473270839117,19.5344432662626,19.6215547336169,19.7086855728379,
19.7604318019191,19.8475621241585,19.9346759052151,20.0217927586668,20.1089048985344,
20.1960364065272,20.2477792996801,20.334905875275,20.4220158905206,20.5091289860856,
20.5962373815785,20.6833651987953,20.7351267974411,20.8222650135847,20.9093867133256,
20.9965114456318,21.0836314228818,21.1707706358326,21.2224742952021,21.3095858066139,
21.396680723011,21.4837788139183,21.570872293834,21.6579854628139,21.7098217929631,
21.7974543214401,21.8850676348139,21.972670334226,21.9911485751285),
 .UNSPECIFIED.);
#1119=B_SPLINE_CURVE_WITH_KNOTS('',3,(#115247,#115248,#115249,#115250,#115251,
#115252,#115253,#115254,#115255,#115256,#115257,#115258,#115259,#115260,
#115261,#115262,#115263,#115264,#115265,#115266,#115267,#115268,#115269,
#115270,#115271,#115272,#115273,#115274,#115275,#115276,#115277,#115278,
#115279,#115280,#115281,#115282,#115283,#115284,#115285,#115286,#115287,
#115288,#115289,#115290,#115291,#115292,#115293,#115294,#115295,#115296,
#115297,#115298,#115299,#115300,#115301,#115302,#115303,#115304,#115305,
#115306,#115307,#115308,#115309,#115310,#115311,#115312,#115313,#115314,
#115315,#115316,#115317,#115318,#115319,#115320,#115321,#115322,#115323,
#115324,#115325,#115326,#115327,#115328,#115329,#115330,#115331,#115332,
#115333,#115334),.UNSPECIFIED.,.F.,.F.,(4,3,3,3,3,3,3,3,3,3,3,3,3,3,3,3,
3,3,3,3,3,3,3,3,3,3,3,3,3,4),(0.,0.0223800438562072,0.0455571551273786,
0.0675550647019532,0.0773342777042101,0.0821512753707187,0.0865889152558688,
0.110577888018856,0.135008177241417,0.157206748761003,0.165672870216831,
0.170323072593406,0.173915834948667,0.198993095015585,0.224022472738064,
0.248522734273473,0.258554636060882,0.264135020452961,0.288903377496841,
0.314991214965926,0.34107905243501,0.351267090483404,0.355315312120404,
0.381664714548266,0.403487578295303,0.410694478291004,0.416463279199868,
0.443066534667852,0.469275862304387,0.472065636590521),.UNSPECIFIED.);
#1120=B_SPLINE_CURVE_WITH_KNOTS('',3,(#115335,#115336,#115337,#115338,#115339,
#115340,#115341,#115342,#115343,#115344,#115345,#115346,#115347,#115348,
#115349,#115350,#115351,#115352,#115353,#115354,#115355,#115356,#115357,
#115358,#115359,#115360,#115361,#115362,#115363,#115364,#115365,#115366,
#115367,#115368,#115369,#115370,#115371,#115372,#115373,#115374,#115375,
#115376,#115377,#115378,#115379,#115380,#115381,#115382,#115383,#115384,
#115385,#115386,#115387,#115388,#115389,#115390,#115391,#115392,#115393,
#115394,#115395,#115396,#115397,#115398,#115399,#115400,#115401,#115402,
#115403,#115404,#115405,#115406,#115407,#115408,#115409,#115410,#115411,
#115412,#115413,#115414,#115415,#115416,#115417,#115418,#115419,#115420,
#115421,#115422),.UNSPECIFIED.,.F.,.F.,(4,3,3,3,3,3,3,3,3,3,3,3,3,3,3,3,
3,3,3,3,3,3,3,3,3,3,3,3,3,4),(0.,0.0260517790363223,0.0527225331664048,
0.0776790837678674,0.0889727987852075,0.0959464344588869,0.100845925000849,
0.126855201330769,0.152534130320941,0.176212520341607,0.186122361847472,
0.192547946339425,0.196620306261614,0.221672219573634,0.246724132885653,
0.272050620367204,0.282513655994357,0.286631738476199,0.311154772354935,
0.33576599459967,0.360166888444423,0.370324933502905,0.375577979330509,
0.399326638864468,0.417608625696714,0.42311115157445,0.427811305959952,
0.450556505121142,0.47164802816755,0.474022601254833),.UNSPECIFIED.);
#1121=B_SPLINE_CURVE_WITH_KNOTS('',3,(#115423,#115424,#115425,#115426,#115427,
#115428,#115429,#115430,#115431,#115432,#115433,#115434,#115435,#115436,
#115437,#115438,#115439,#115440,#115441,#115442,#115443,#115444,#115445,
#115446,#115447,#115448,#115449,#115450,#115451,#115452,#115453,#115454,
#115455,#115456,#115457,#115458,#115459,#115460,#115461,#115462,#115463,
#115464,#115465,#115466,#115467,#115468,#115469,#115470,#115471,#115472,
#115473,#115474,#115475,#115476,#115477,#115478,#115479,#115480,#115481,
#115482,#115483,#115484,#115485,#115486,#115487,#115488,#115489,#115490,
#115491,#115492,#115493,#115494,#115495,#115496,#115497,#115498,#115499,
#115500,#115501,#115502,#115503,#115504,#115505,#115506,#115507,#115508,
#115509,#115510),.UNSPECIFIED.,.F.,.F.,(4,3,3,3,3,3,3,3,3,3,3,3,3,3,3,3,
3,3,3,3,3,3,3,3,3,3,3,3,3,4),(0.,0.0223800372151316,0.0455571433117667,
0.0675550536686484,0.0773342673604862,0.0821512524289193,0.0865889078224679,
0.110577875996278,0.135008164712988,0.157206738276085,0.165672856963219,
0.170323012283074,0.173915733667268,0.198992994974291,0.224022472738052,
0.248477225379953,0.258554635842646,0.264135020504929,0.288903381765904,
0.314991218209838,0.341079054653772,0.351267092682162,0.355315313446979,
0.38166471636314,0.403487580067799,0.410694485847216,0.41646327764549,0.443066533245085,
0.469275862304372,0.472065636984189),.UNSPECIFIED.);
#1122=B_SPLINE_CURVE_WITH_KNOTS('',3,(#115511,#115512,#115513,#115514,#115515,
#115516,#115517,#115518,#115519,#115520,#115521,#115522,#115523,#115524,
#115525,#115526,#115527,#115528,#115529,#115530,#115531,#115532,#115533,
#115534,#115535,#115536,#115537,#115538,#115539,#115540,#115541,#115542,
#115543,#115544,#115545,#115546,#115547,#115548,#115549,#115550,#115551,
#115552,#115553,#115554,#115555,#115556,#115557,#115558,#115559,#115560,
#115561,#115562,#115563,#115564,#115565,#115566,#115567,#115568,#115569,
#115570,#115571,#115572,#115573,#115574,#115575,#115576,#115577,#115578,
#115579,#115580,#115581,#115582,#115583,#115584,#115585,#115586,#115587,
#115588,#115589,#115590,#115591,#115592,#115593,#115594,#115595,#115596,
#115597,#115598),.UNSPECIFIED.,.F.,.F.,(4,3,3,3,3,3,3,3,3,3,3,3,3,3,3,3,
3,3,3,3,3,3,3,3,3,3,3,3,3,4),(0.,0.026051796848667,0.0527225544334848,0.0776790985121134,
0.088972803707389,0.0959464341599202,0.100845925569268,0.126855201703197,
0.152534124110727,0.176212516457141,0.186122361672799,0.192547951517572,
0.196620308043645,0.221672220464654,0.246724132885662,0.272050621021719,
0.282513655344617,0.286631737801889,0.311154771378495,0.335765992433512,
0.360166881962943,0.370324927588301,0.375577975882316,0.399326629362454,
0.417608623757103,0.423111147264353,0.427811294162416,0.4505564811234,0.471648028167544,
0.474022601254839),.UNSPECIFIED.);
#1123=B_SPLINE_CURVE_WITH_KNOTS('',3,(#115599,#115600,#115601,#115602,#115603,
#115604,#115605,#115606,#115607,#115608,#115609,#115610,#115611,#115612,
#115613,#115614,#115615,#115616,#115617,#115618,#115619,#115620,#115621,
#115622,#115623,#115624,#115625,#115626,#115627,#115628,#115629,#115630,
#115631,#115632,#115633,#115634,#115635,#115636,#115637,#115638,#115639,
#115640,#115641,#115642,#115643,#115644,#115645,#115646,#115647,#115648,
#115649,#115650,#115651,#115652,#115653,#115654,#115655,#115656,#115657,
#115658,#115659,#115660,#115661,#115662,#115663,#115664,#115665,#115666,
#115667,#115668,#115669,#115670,#115671,#115672,#115673,#115674,#115675,
#115676,#115677,#115678,#115679,#115680,#115681,#115682,#115683,#115684,
#115685,#115686),.UNSPECIFIED.,.F.,.F.,(4,3,3,3,3,3,3,3,3,3,3,3,3,3,3,3,
3,3,3,3,3,3,3,3,3,3,3,3,3,4),(0.,0.0226012852117639,0.0452025704235279,
0.067555058212843,0.0773342716206684,0.0821512618789957,0.0865889109720383,
0.110761871811172,0.134934832650306,0.157206742672241,0.165672862519276,
0.17032303759631,0.173915776335193,0.198993037124028,0.224022472738049,
0.24847722404691,0.258554635931002,0.264135020402494,0.289777625640233,
0.315428339653183,0.341079053666132,0.351267091758101,0.355315312641973,
0.381664715351709,0.403487579124147,0.410694481959163,0.416463278906866,
0.443066534477177,0.469275862304408,0.472065636821688),.UNSPECIFIED.);
#1124=B_SPLINE_CURVE_WITH_KNOTS('',3,(#115687,#115688,#115689,#115690,#115691,
#115692,#115693,#115694,#115695,#115696,#115697,#115698,#115699,#115700,
#115701,#115702,#115703,#115704,#115705,#115706,#115707,#115708,#115709,
#115710,#115711,#115712,#115713,#115714,#115715,#115716,#115717,#115718,
#115719,#115720,#115721,#115722,#115723,#115724,#115725,#115726,#115727,
#115728,#115729,#115730,#115731,#115732,#115733,#115734,#115735,#115736,
#115737,#115738,#115739,#115740,#115741,#115742,#115743,#115744,#115745,
#115746,#115747,#115748,#115749,#115750,#115751,#115752,#115753,#115754,
#115755,#115756,#115757,#115758,#115759,#115760,#115761,#115762,#115763,
#115764,#115765,#115766,#115767,#115768,#115769,#115770,#115771,#115772,
#115773,#115774),.UNSPECIFIED.,.F.,.F.,(4,3,3,3,3,3,3,3,3,3,3,3,3,3,3,3,
3,3,3,3,3,3,3,3,3,3,3,3,3,4),(0.,0.0259306190073998,0.0526009583628531,
0.0776790988226147,0.0889728038113335,0.0959464341623167,0.100845925575729,
0.126856858203816,0.152713971434144,0.177949842661195,0.186122361669415,
0.192547951595364,0.196620308076219,0.221672220480934,0.24672413288565,
0.272050621046898,0.282513655340624,0.286631737980665,0.311197491830502,
0.335883934797747,0.360158613793621,0.3703249274938,0.375577975829039,0.399326629202052,
0.41760862372711,0.423111147116857,0.427811294064984,0.450556480771393,
0.471648028167486,0.47402260125479),.UNSPECIFIED.);
#1125=B_SPLINE_CURVE_WITH_KNOTS('',3,(#115775,#115776,#115777,#115778,#115779,
#115780,#115781,#115782,#115783,#115784,#115785,#115786,#115787,#115788,
#115789,#115790,#115791,#115792,#115793,#115794,#115795,#115796,#115797,
#115798,#115799,#115800,#115801,#115802,#115803,#115804,#115805,#115806,
#115807,#115808,#115809,#115810,#115811,#115812,#115813,#115814,#115815,
#115816,#115817,#115818,#115819,#115820,#115821,#115822,#115823,#115824,
#115825,#115826,#115827,#115828,#115829,#115830,#115831,#115832,#115833,
#115834,#115835,#115836,#115837,#115838,#115839,#115840,#115841,#115842,
#115843,#115844,#115845,#115846,#115847,#115848,#115849,#115850,#115851,
#115852,#115853,#115854,#115855,#115856,#115857,#115858,#115859,#115860,
#115861,#115862),.UNSPECIFIED.,.F.,.F.,(4,3,3,3,3,3,3,3,3,3,3,3,3,3,3,3,
3,3,3,3,3,3,3,3,3,3,3,3,3,4),(0.,0.0223800600970211,0.0455571838797127,
0.0675550913477831,0.0773343026846742,0.0821513307715598,0.086588933128813,
0.110761903794659,0.134934874460505,0.159278641767769,0.165672902158484,
0.170323218744956,0.173916080012127,0.198993337115258,0.224022472738042,
0.248522726826221,0.25855463659488,0.264135020001501,0.288903366541003,
0.314991206662608,0.341079046784212,0.351267085078404,0.355315309150301,
0.381664710560743,0.403487574104964,0.411770819428486,0.416463283580499,
0.443066538814217,0.469275862304419,0.472065635637229),.UNSPECIFIED.);
#1126=B_SPLINE_CURVE_WITH_KNOTS('',3,(#115863,#115864,#115865,#115866,#115867,
#115868,#115869,#115870,#115871,#115872,#115873,#115874,#115875,#115876,
#115877,#115878,#115879,#115880,#115881,#115882,#115883,#115884,#115885,
#115886,#115887,#115888,#115889,#115890,#115891,#115892,#115893,#115894,
#115895,#115896,#115897,#115898,#115899,#115900,#115901,#115902,#115903,
#115904,#115905,#115906,#115907,#115908,#115909,#115910,#115911,#115912,
#115913,#115914,#115915,#115916,#115917,#115918,#115919,#115920,#115921,
#115922,#115923,#115924,#115925,#115926,#115927,#115928,#115929,#115930,
#115931,#115932,#115933,#115934,#115935,#115936,#115937,#115938,#115939,
#115940,#115941,#115942,#115943,#115944,#115945,#115946,#115947),
 .UNSPECIFIED.,.F.,.F.,(4,3,3,3,3,3,3,3,3,3,3,3,3,3,3,3,3,3,3,3,3,3,3,3,
3,3,3,3,4),(0.,0.0260517912929958,0.0527225478357444,0.0776790939050551,
0.0889728021702812,0.0959464342551659,0.100845925350706,0.126855201462979,
0.152534125915518,0.176212517636641,0.192547949849574,0.196620307478408,
0.221672220182029,0.24672413288565,0.272050620811562,0.282513655553444,
0.286631738154676,0.311154771782915,0.335765993221651,0.360166884129707,
0.370324929459797,0.375577976970675,0.399326632351765,0.417608624369275,
0.423111148621278,0.427811298126592,0.450556488913048,0.471648028167475,
0.474022601254778),.UNSPECIFIED.);
#1127=B_SPLINE_CURVE_WITH_KNOTS('',3,(#116164,#116165,#116166,#116167,#116168,
#116169,#116170,#116171,#116172,#116173,#116174,#116175,#116176,#116177,
#116178,#116179,#116180,#116181,#116182,#116183,#116184,#116185,#116186,
#116187,#116188,#116189,#116190,#116191,#116192,#116193,#116194,#116195,
#116196,#116197,#116198,#116199,#116200,#116201,#116202,#116203,#116204,
#116205,#116206,#116207,#116208,#116209,#116210,#116211,#116212,#116213,
#116214,#116215,#116216,#116217,#116218,#116219,#116220,#116221,#116222,
#116223,#116224,#116225,#116226,#116227,#116228,#116229,#116230,#116231,
#116232,#116233,#116234,#116235,#116236,#116237,#116238,#116239,#116240,
#116241,#116242,#116243,#116244,#116245,#116246,#116247,#116248,#116249,
#116250,#116251,#116252,#116253,#116254,#116255,#116256,#116257,#116258,
#116259,#116260,#116261,#116262,#116263,#116264,#116265,#116266),
 .UNSPECIFIED.,.F.,.F.,(4,3,3,3,3,3,3,3,3,3,3,3,3,3,3,3,3,3,3,3,3,3,3,3,
3,3,3,3,3,3,3,3,3,3,4),(-0.950777871811442,-0.906336425390159,-0.861875033089073,
-0.842434685731619,-0.832698894406312,-0.823679279214301,-0.779911530229351,
-0.736812975210593,-0.713111655774817,-0.707528734983928,-0.706840830508988,
-0.663970529007278,-0.620960197429003,-0.578452544067916,-0.53653757030824,
-0.528618153061017,-0.519778489990599,-0.479103795974014,-0.472085166836762,
-0.430141730544586,-0.388512020620237,-0.35295009564229,-0.345831806228506,
-0.34009678874744,-0.299353453374951,-0.258818746671375,-0.246812444972861,
-0.206136253916918,-0.172639040264036,-0.165053203014642,-0.125295016427035,
-0.0858747403745168,-0.046745972523297,-0.0311581910594031,0.),
 .UNSPECIFIED.);
#1128=B_SPLINE_CURVE_WITH_KNOTS('',3,(#116267,#116268,#116269,#116270,#116271,
#116272,#116273,#116274,#116275,#116276,#116277,#116278,#116279,#116280,
#116281,#116282,#116283,#116284,#116285,#116286,#116287,#116288,#116289,
#116290,#116291,#116292,#116293,#116294,#116295,#116296,#116297,#116298,
#116299,#116300,#116301,#116302,#116303,#116304,#116305,#116306,#116307,
#116308,#116309,#116310,#116311,#116312,#116313,#116314,#116315,#116316,
#116317,#116318,#116319,#116320,#116321,#116322,#116323,#116324,#116325,
#116326,#116327,#116328,#116329,#116330,#116331,#116332,#116333,#116334,
#116335,#116336,#116337,#116338,#116339,#116340,#116341,#116342,#116343,
#116344,#116345,#116346,#116347,#116348,#116349,#116350,#116351,#116352,
#116353,#116354,#116355,#116356,#116357,#116358,#116359,#116360,#116361,
#116362,#116363,#116364,#116365,#116366,#116367,#116368,#116369),
 .UNSPECIFIED.,.F.,.F.,(4,3,3,3,3,3,3,3,3,3,3,3,3,3,3,3,3,3,3,3,3,3,3,3,
3,3,3,3,3,3,3,3,3,3,4),(0.,0.0392937243200445,0.0786487924196305,0.118430422481545,
0.157174897280178,0.16530965460934,0.172511921016207,0.214141585432509,
0.254364238175761,0.295024495339404,0.33584270732332,0.340554091141284,
0.347540360366197,0.389002662438925,0.430931272522026,0.437981494075935,
0.479749916301,0.518812960683757,0.524399035770372,0.530138494511844,0.572626647084422,
0.615529815031132,0.658476413958322,0.671400602336179,0.691337520740504,
0.703515645425686,0.711692863472691,0.721145455869737,0.764504689598731,
0.808363873661209,0.829117588621419,0.836453781446258,0.880985314545995,
0.913941349417081,0.950775682567348),.UNSPECIFIED.);
#1129=B_SPLINE_CURVE_WITH_KNOTS('',3,(#116586,#116587,#116588,#116589,#116590,
#116591,#116592,#116593,#116594,#116595,#116596,#116597,#116598,#116599,
#116600,#116601,#116602,#116603,#116604,#116605,#116606,#116607,#116608,
#116609,#116610,#116611,#116612,#116613,#116614,#116615,#116616,#116617,
#116618,#116619,#116620,#116621,#116622,#116623,#116624,#116625,#116626,
#116627,#116628,#116629,#116630,#116631,#116632,#116633,#116634,#116635,
#116636,#116637,#116638,#116639,#116640,#116641,#116642,#116643,#116644,
#116645,#116646,#116647,#116648,#116649,#116650,#116651,#116652,#116653,
#116654,#116655,#116656,#116657,#116658,#116659,#116660,#116661,#116662,
#116663,#116664,#116665,#116666,#116667,#116668,#116669,#116670,#116671,
#116672,#116673,#116674,#116675,#116676,#116677,#116678,#116679,#116680,
#116681,#116682,#116683,#116684,#116685),.UNSPECIFIED.,.F.,.F.,(4,3,3,3,
3,3,3,3,3,3,3,3,3,3,3,3,3,3,3,3,3,3,3,3,3,3,3,3,3,3,3,3,3,4),(-0.954382097139067,
-0.915540356901116,-0.875987953894438,-0.858553371309591,-0.851652578164575,
-0.844316096216611,-0.803953485084634,-0.771951682750547,-0.755904221756574,
-0.746876223962411,-0.741004834362442,-0.7398567607626,-0.698120295630557,
-0.65723238014393,-0.615071640189179,-0.572910900234428,-0.567449445615807,
-0.525372539405531,-0.515246554457167,-0.473498151147521,-0.43027138546824,
-0.387044619788958,-0.380028835389925,-0.33707776560403,-0.293664876803929,
-0.280914982302858,-0.237661647632792,-0.200416680658377,-0.194604991995093,
-0.150716444031498,-0.106377373616171,-0.0619596473153769,-0.0369876293288037,
-2.19658856801564E-6),.UNSPECIFIED.);
#1130=B_SPLINE_CURVE_WITH_KNOTS('',3,(#116686,#116687,#116688,#116689,#116690,
#116691,#116692,#116693,#116694,#116695,#116696,#116697,#116698,#116699,
#116700,#116701,#116702,#116703,#116704,#116705,#116706,#116707,#116708,
#116709,#116710,#116711,#116712,#116713,#116714,#116715,#116716,#116717,
#116718,#116719,#116720,#116721,#116722,#116723,#116724,#116725,#116726,
#116727,#116728,#116729,#116730,#116731,#116732,#116733,#116734,#116735,
#116736,#116737,#116738,#116739,#116740,#116741,#116742,#116743,#116744,
#116745,#116746,#116747,#116748,#116749,#116750,#116751,#116752,#116753,
#116754,#116755,#116756,#116757,#116758,#116759,#116760,#116761,#116762,
#116763,#116764,#116765,#116766,#116767,#116768,#116769,#116770,#116771,
#116772,#116773,#116774,#116775,#116776,#116777,#116778,#116779,#116780,
#116781,#116782,#116783,#116784,#116785,#116786,#116787,#116788),
 .UNSPECIFIED.,.F.,.F.,(4,3,3,3,3,3,3,3,3,3,3,3,3,3,3,3,3,3,3,3,3,3,3,3,
3,3,3,3,3,3,3,3,3,3,4),(3.92004242434274E-15,0.0440097382289256,0.0884882554294149,
0.132783546544066,0.176334546385407,0.187993870420512,0.19423572748739,
0.19979115047153,0.245254179237364,0.288657155098447,0.331818541229242,
0.369239411527086,0.3808541168619,0.388821225436964,0.431108255685869,0.473065176330631,
0.481013297040258,0.523218576167236,0.558979311157592,0.56811322256641,
0.573516263988367,0.614763363362679,0.655642090780445,0.696286761208482,
0.70713567464641,0.734136415169824,0.744264975553648,0.750002339682418,
0.790439331413101,0.830523899179901,0.849662847172381,0.855799185905343,
0.89514518435056,0.923141598833727,0.954382097139069),.UNSPECIFIED.);
#1131=B_SPLINE_CURVE_WITH_KNOTS('',3,(#117005,#117006,#117007,#117008,#117009,
#117010,#117011,#117012,#117013,#117014,#117015,#117016,#117017,#117018,
#117019,#117020,#117021,#117022,#117023,#117024,#117025,#117026,#117027,
#117028,#117029,#117030,#117031,#117032,#117033,#117034,#117035,#117036,
#117037,#117038,#117039,#117040,#117041,#117042,#117043,#117044,#117045,
#117046,#117047,#117048,#117049,#117050,#117051,#117052,#117053,#117054,
#117055,#117056,#117057,#117058,#117059,#117060,#117061,#117062,#117063,
#117064,#117065,#117066,#117067,#117068,#117069,#117070,#117071,#117072,
#117073,#117074,#117075,#117076,#117077,#117078,#117079,#117080,#117081,
#117082,#117083,#117084,#117085,#117086,#117087,#117088,#117089,#117090,
#117091,#117092,#117093,#117094,#117095,#117096,#117097,#117098,#117099,
#117100,#117101,#117102,#117103,#117104,#117105,#117106,#117107,#117108,
#117109,#117110),.UNSPECIFIED.,.F.,.F.,(4,3,3,3,3,3,3,3,3,3,3,3,3,3,3,3,
3,3,3,3,3,3,3,3,3,3,3,3,3,3,3,3,3,3,3,4),(-0.950777871811489,-0.906336436543847,
-0.861875037007214,-0.842434689817133,-0.831093639563838,-0.825301574638444,
-0.781525133147754,-0.738411526679266,-0.713111654821142,-0.707528734408151,
-0.70684083050903,-0.664137304886555,-0.621129293429489,-0.578512194042679,
-0.536486363527969,-0.527113745436322,-0.519453631979133,-0.479103798452372,
-0.472085166836776,-0.430141731436697,-0.388512022347839,-0.352950096664573,
-0.345831809185344,-0.340096789032849,-0.299287338987684,-0.258818748563885,
-0.246812444972867,-0.206034245191202,-0.184174738424728,-0.172639040064828,
-0.16435164756875,-0.124589561125894,-0.0849805995896592,-0.0460567214496698,
-0.0311581910594067,0.),.UNSPECIFIED.);
#1132=B_SPLINE_CURVE_WITH_KNOTS('',3,(#117111,#117112,#117113,#117114,#117115,
#117116,#117117,#117118,#117119,#117120,#117121,#117122,#117123,#117124,
#117125,#117126,#117127,#117128,#117129,#117130,#117131,#117132,#117133,
#117134,#117135,#117136,#117137,#117138,#117139,#117140,#117141,#117142,
#117143,#117144,#117145,#117146,#117147,#117148,#117149,#117150,#117151,
#117152,#117153,#117154,#117155,#117156,#117157,#117158,#117159,#117160,
#117161,#117162,#117163,#117164,#117165,#117166,#117167,#117168,#117169,
#117170,#117171,#117172,#117173,#117174,#117175,#117176,#117177,#117178,
#117179,#117180,#117181,#117182,#117183,#117184,#117185,#117186,#117187,
#117188,#117189,#117190,#117191,#117192,#117193,#117194,#117195,#117196,
#117197,#117198,#117199,#117200,#117201,#117202,#117203,#117204,#117205,
#117206,#117207,#117208,#117209,#117210,#117211,#117212,#117213),
 .UNSPECIFIED.,.F.,.F.,(4,3,3,3,3,3,3,3,3,3,3,3,3,3,3,3,3,3,3,3,3,3,3,3,
3,3,3,3,3,3,3,3,3,3,4),(2.82530270380345E-15,0.0383561142044287,0.0777322538494532,
0.117448352722929,0.157136327544403,0.16530959676955,0.172511917896846,
0.214141585432506,0.254319391003506,0.295111323821477,0.330724243378432,
0.341693770779803,0.34884651352764,0.390592332836265,0.430931232999916,
0.437981494075929,0.47974991115956,0.518812944385605,0.524709771531363,
0.530138484534004,0.572570423222228,0.615574325973383,0.658476390767529,
0.671400602336174,0.701718195721287,0.711077059751642,0.717874112270349,
0.761139330498555,0.804963166413865,0.816774798744654,0.829117599322156,
0.836453798394249,0.880985331409101,0.913941349417075,0.950775682377206),
 .UNSPECIFIED.);
#1133=B_SPLINE_CURVE_WITH_KNOTS('',3,(#117430,#117431,#117432,#117433,#117434,
#117435,#117436,#117437,#117438,#117439,#117440,#117441,#117442,#117443,
#117444,#117445,#117446,#117447,#117448,#117449,#117450,#117451,#117452,
#117453,#117454,#117455,#117456,#117457,#117458,#117459,#117460,#117461,
#117462,#117463,#117464,#117465,#117466,#117467,#117468,#117469,#117470,
#117471,#117472,#117473,#117474,#117475,#117476,#117477,#117478,#117479,
#117480,#117481,#117482,#117483,#117484,#117485,#117486,#117487,#117488,
#117489,#117490,#117491,#117492,#117493,#117494,#117495,#117496,#117497,
#117498,#117499,#117500,#117501,#117502,#117503,#117504,#117505,#117506,
#117507,#117508,#117509,#117510,#117511,#117512,#117513,#117514,#117515,
#117516,#117517,#117518,#117519,#117520,#117521,#117522,#117523,#117524,
#117525,#117526,#117527,#117528,#117529,#117530,#117531,#117532,#117533,
#117534,#117535),.UNSPECIFIED.,.F.,.F.,(4,3,3,3,3,3,3,3,3,3,3,3,3,3,3,3,
3,3,3,3,3,3,3,3,3,3,3,3,3,3,3,3,3,3,3,4),(-0.954382097139027,-0.915540393312973,
-0.875988011034615,-0.858553452015747,-0.851651720979109,-0.84431594622701,
-0.803953347308937,-0.771951616163724,-0.755904188463154,-0.746876173424658,
-0.741004793318458,-0.739856760762583,-0.698120275698938,-0.657232336987902,
-0.615071578747952,-0.572910820508001,-0.567449396059044,-0.525372472030206,
-0.515246554457162,-0.473526932909519,-0.431236741000685,-0.393744912161324,
-0.387044679913831,-0.381221890286597,-0.338027165363517,-0.294874550582207,
-0.28091498230286,-0.237709647788546,-0.212648675820495,-0.200416680015836,
-0.194604990965853,-0.150716441724809,-0.106377371179378,-0.0619596447542818,
-0.0369876293288071,-2.19683063229992E-6),.UNSPECIFIED.);
#1134=B_SPLINE_CURVE_WITH_KNOTS('',3,(#117536,#117537,#117538,#117539,#117540,
#117541,#117542,#117543,#117544,#117545,#117546,#117547,#117548,#117549,
#117550,#117551,#117552,#117553,#117554,#117555,#117556,#117557,#117558,
#117559,#117560,#117561,#117562,#117563,#117564,#117565,#117566,#117567,
#117568,#117569,#117570,#117571,#117572,#117573,#117574,#117575,#117576,
#117577,#117578,#117579,#117580,#117581,#117582,#117583,#117584,#117585,
#117586,#117587,#117588,#117589,#117590,#117591,#117592,#117593,#117594,
#117595,#117596,#117597,#117598,#117599,#117600,#117601,#117602,#117603,
#117604,#117605,#117606,#117607,#117608,#117609,#117610,#117611,#117612,
#117613,#117614,#117615,#117616,#117617,#117618,#117619,#117620,#117621,
#117622,#117623,#117624,#117625,#117626,#117627,#117628,#117629,#117630,
#117631,#117632,#117633,#117634,#117635,#117636,#117637,#117638,#117639,
#117640,#117641),.UNSPECIFIED.,.F.,.F.,(4,3,3,3,3,3,3,3,3,3,3,3,3,3,3,3,
3,3,3,3,3,3,3,3,3,3,3,3,3,3,3,3,3,3,3,4),(0.,0.0440097102619092,0.0884882277676935,
0.13278353303231,0.176334557243214,0.187993903233133,0.194235848510683,
0.199791297605252,0.245254179237363,0.288657161367,0.331818543101246,0.369239414789171,
0.380854128970053,0.388821223648941,0.43103452325887,0.473065169701532,
0.481013297040253,0.523218575748239,0.558979309133477,0.568113222474232,
0.57351626392526,0.614765000689446,0.655861440304519,0.69628675606685,0.707135674646407,
0.734136415169823,0.74426497460981,0.752455611723686,0.792892563016178,
0.833036427742995,0.838982768060298,0.849662831772539,0.855799161052988,
0.895145162238262,0.923141598833728,0.954382097139071),.UNSPECIFIED.);
#1135=B_SPLINE_CURVE_WITH_KNOTS('',3,(#118354,#118355,#118356,#118357,#118358,
#118359,#118360,#118361,#118362,#118363,#118364,#118365,#118366,#118367,
#118368,#118369,#118370,#118371,#118372,#118373,#118374,#118375,#118376,
#118377,#118378,#118379,#118380,#118381,#118382,#118383,#118384,#118385,
#118386,#118387,#118388,#118389,#118390,#118391,#118392,#118393,#118394,
#118395,#118396,#118397,#118398,#118399,#118400,#118401,#118402,#118403,
#118404,#118405,#118406,#118407,#118408,#118409,#118410,#118411,#118412,
#118413,#118414,#118415,#118416,#118417,#118418,#118419,#118420,#118421,
#118422,#118423,#118424,#118425,#118426,#118427,#118428,#118429,#118430,
#118431,#118432,#118433,#118434,#118435,#118436,#118437,#118438,#118439,
#118440,#118441),.UNSPECIFIED.,.F.,.F.,(4,3,3,3,3,3,3,3,3,3,3,3,3,3,3,3,
3,3,3,3,3,3,3,3,3,3,3,3,3,4),(0.,0.0223800415826112,0.0455571510727117,
0.0675550609170155,0.0773342741558292,0.0821512675008773,0.0865889126878389,
0.110577883862217,0.13500817294145,0.157206745152612,0.16567286565653,0.170323051943897,
0.173915800266865,0.198993060769187,0.224022472738035,0.248477223249604,
0.258554635986008,0.264135020444879,0.288903378930059,0.314991216050641,
0.341079053171223,0.351267091230857,0.355315312478378,0.381664715071333,
0.403487578818942,0.410694480570935,0.416463278950785,0.443066534470942,
0.469275862304353,0.472065636725432),.UNSPECIFIED.);
#1136=B_SPLINE_CURVE_WITH_KNOTS('',3,(#119154,#119155,#119156,#119157,#119158,
#119159,#119160,#119161,#119162,#119163,#119164,#119165,#119166,#119167,
#119168,#119169,#119170,#119171,#119172,#119173,#119174,#119175,#119176,
#119177,#119178,#119179,#119180,#119181,#119182,#119183,#119184,#119185,
#119186,#119187,#119188,#119189,#119190,#119191,#119192,#119193,#119194,
#119195,#119196,#119197,#119198,#119199,#119200,#119201,#119202,#119203,
#119204,#119205,#119206,#119207,#119208,#119209,#119210,#119211,#119212,
#119213,#119214,#119215,#119216,#119217,#119218,#119219,#119220,#119221,
#119222,#119223,#119224,#119225,#119226,#119227,#119228,#119229,#119230,
#119231,#119232,#119233,#119234,#119235,#119236,#119237,#119238,#119239,
#119240,#119241,#119242,#119243,#119244),.UNSPECIFIED.,.F.,.F.,(4,3,3,3,
3,3,3,3,3,3,3,3,3,3,3,3,3,3,3,3,3,3,3,3,3,3,3,3,3,3,4),(7.90123170449159E-15,
0.026051780813598,0.0527225352993908,0.0776790852361114,0.0889727992741923,
0.0959464344241781,0.100845925040092,0.126855201361833,0.152534129666993,
0.17621251994363,0.186122361828502,0.19254794682658,0.196620306433238,0.221672219659448,
0.246724132885659,0.27205844796921,0.280886246323336,0.285802388621783,
0.299566540225716,0.311229550951507,0.335915922421445,0.36019020093975,
0.370324932919906,0.375577978970566,0.399326637919176,0.417608625494232,
0.423111151172439,0.427811304835429,0.450556502779003,0.471648028167516,
0.474022601254811),.UNSPECIFIED.);
#1137=B_SPLINE_CURVE_WITH_KNOTS('',3,(#119957,#119958,#119959,#119960,#119961,
#119962,#119963,#119964,#119965,#119966,#119967,#119968,#119969,#119970,
#119971,#119972,#119973,#119974,#119975,#119976,#119977,#119978,#119979,
#119980,#119981,#119982,#119983,#119984,#119985,#119986,#119987,#119988,
#119989,#119990,#119991,#119992,#119993,#119994,#119995,#119996,#119997,
#119998,#119999,#120000,#120001,#120002,#120003,#120004,#120005,#120006,
#120007,#120008,#120009,#120010,#120011,#120012,#120013,#120014,#120015,
#120016,#120017,#120018,#120019,#120020,#120021,#120022,#120023,#120024,
#120025,#120026,#120027,#120028,#120029,#120030,#120031,#120032,#120033,
#120034,#120035,#120036,#120037,#120038,#120039,#120040,#120041,#120042,
#120043,#120044),.UNSPECIFIED.,.F.,.F.,(4,3,3,3,3,3,3,3,3,3,3,3,3,3,3,3,
3,3,3,3,3,3,3,3,3,3,3,3,3,4),(0.,0.0223800646564789,0.0455571919885243,
0.0675550989125488,0.077334309776642,0.0821513465008637,0.0865889382889745,
0.110577925353256,0.135008216272887,0.157206781258753,0.165672911295151,
0.170323260534971,0.173916149941423,0.198993406189961,0.22402247273804,
0.248477212094458,0.258554636746328,0.26413501995488,0.288903363466093,
0.314991204360096,0.341079045254099,0.351267083567837,0.355315308310309,
0.381664709440851,0.403487572943969,0.410694455370546,0.416463284762423,
0.443066539898885,0.469275862304369,0.472065635365967),.UNSPECIFIED.);
#1138=B_SPLINE_CURVE_WITH_KNOTS('',3,(#120757,#120758,#120759,#120760,#120761,
#120762,#120763,#120764,#120765,#120766,#120767,#120768,#120769,#120770,
#120771,#120772,#120773,#120774,#120775,#120776,#120777,#120778,#120779,
#120780,#120781,#120782,#120783,#120784,#120785,#120786,#120787,#120788,
#120789,#120790,#120791,#120792,#120793,#120794,#120795,#120796,#120797,
#120798,#120799,#120800,#120801,#120802,#120803,#120804,#120805,#120806,
#120807,#120808,#120809,#120810,#120811,#120812,#120813,#120814,#120815,
#120816,#120817,#120818,#120819,#120820,#120821,#120822,#120823,#120824,
#120825,#120826,#120827,#120828,#120829,#120830,#120831,#120832,#120833,
#120834,#120835,#120836,#120837,#120838,#120839,#120840,#120841,#120842,
#120843,#120844),.UNSPECIFIED.,.F.,.F.,(4,3,3,3,3,3,3,3,3,3,3,3,3,3,3,3,
3,3,3,3,3,3,3,3,3,3,3,3,3,4),(0.,0.0260517756043454,0.052722529084373,0.0776790809548157,
0.0889727978441528,0.0959464345074647,0.10084592486155,0.126855201263957,
0.152534131466515,0.176212521061365,0.186122361876941,0.192547945329784,
0.196620305916515,0.221672219401092,0.246724132885669,0.27206158277579,
0.282513656118586,0.286631738568381,0.311197492372782,0.335883935060444,
0.360158620946212,0.370324934628168,0.375577979963716,0.399595492014671,
0.417608626052888,0.423111152459427,0.427811308268704,0.450556509740111,
0.471648028167537,0.474022601254832),.UNSPECIFIED.);
#1139=B_SPLINE_CURVE_WITH_KNOTS('',3,(#121557,#121558,#121559,#121560,#121561,
#121562,#121563,#121564,#121565,#121566,#121567,#121568,#121569,#121570,
#121571,#121572,#121573,#121574,#121575,#121576,#121577,#121578,#121579,
#121580,#121581,#121582,#121583,#121584,#121585,#121586,#121587,#121588,
#121589,#121590,#121591,#121592,#121593,#121594,#121595,#121596,#121597,
#121598,#121599,#121600,#121601,#121602,#121603,#121604,#121605,#121606,
#121607,#121608,#121609,#121610,#121611,#121612,#121613,#121614,#121615,
#121616,#121617,#121618,#121619,#121620,#121621,#121622,#121623,#121624,
#121625,#121626,#121627,#121628,#121629,#121630,#121631,#121632,#121633,
#121634,#121635,#121636,#121637,#121638,#121639,#121640,#121641,#121642,
#121643,#121644),.UNSPECIFIED.,.F.,.F.,(4,3,3,3,3,3,3,3,3,3,3,3,3,3,3,3,
3,3,3,3,3,3,3,3,3,3,3,3,3,4),(0.,0.0223800651370379,0.0455571928568217,
0.0675550997304994,0.0773343105434705,0.0833848318194915,0.0865889388358174,
0.110577926266236,0.135008217226719,0.157206782032257,0.165672912272975,
0.170323265017005,0.173916157466764,0.198993413622444,0.224022472738036,
0.248477211854248,0.258554636762497,0.264135019948427,0.288981342589089,
0.314338830546098,0.340111642434369,0.351267083403808,0.355315308234309,
0.381664709331106,0.403487572828058,0.410694454865743,0.416463284884501,
0.443066539997531,0.469275862304369,0.472065635336616),.UNSPECIFIED.);
#1140=B_SPLINE_CURVE_WITH_KNOTS('',3,(#122357,#122358,#122359,#122360,#122361,
#122362,#122363,#122364,#122365,#122366,#122367,#122368,#122369,#122370,
#122371,#122372,#122373,#122374,#122375,#122376,#122377,#122378,#122379,
#122380,#122381,#122382,#122383,#122384,#122385,#122386,#122387,#122388,
#122389,#122390,#122391,#122392,#122393,#122394,#122395,#122396,#122397,
#122398,#122399,#122400,#122401,#122402,#122403,#122404,#122405,#122406,
#122407,#122408,#122409,#122410,#122411,#122412,#122413,#122414,#122415,
#122416,#122417,#122418,#122419,#122420,#122421,#122422,#122423,#122424,
#122425,#122426,#122427,#122428,#122429,#122430,#122431,#122432,#122433,
#122434,#122435,#122436,#122437,#122438,#122439,#122440,#122441,#122442,
#122443,#122444),.UNSPECIFIED.,.F.,.F.,(4,3,3,3,3,3,3,3,3,3,3,3,3,3,3,3,
3,3,3,3,3,3,3,3,3,3,3,3,3,4),(0.,0.0261324658014225,0.0526962913265927,
0.079341535722988,0.0889727984346616,0.0958350432501777,0.10084592493607,
0.126856858695131,0.152713978118554,0.177949856032678,0.186122361857045,
0.192547945950156,0.196620306130287,0.221672219507975,0.246724132885664,
0.272050620322494,0.282513656041832,0.286631738502527,0.311258832154326,
0.335885925806125,0.360166888882926,0.37032493392055,0.375577979558784,
0.399326639542125,0.417608625825101,0.423111151926387,0.42781130682219,
0.450556506836619,0.47164802816751,0.474022601254803),.UNSPECIFIED.);
#1141=B_SPLINE_CURVE_WITH_KNOTS('',3,(#123157,#123158,#123159,#123160,#123161,
#123162,#123163,#123164,#123165,#123166,#123167,#123168,#123169,#123170,
#123171,#123172,#123173,#123174,#123175,#123176,#123177,#123178,#123179,
#123180,#123181,#123182,#123183,#123184,#123185,#123186,#123187,#123188,
#123189,#123190,#123191,#123192,#123193,#123194,#123195,#123196,#123197,
#123198,#123199,#123200,#123201,#123202,#123203,#123204,#123205,#123206,
#123207,#123208,#123209,#123210,#123211,#123212,#123213,#123214,#123215,
#123216,#123217,#123218,#123219,#123220,#123221,#123222,#123223,#123224,
#123225,#123226,#123227,#123228,#123229,#123230,#123231,#123232,#123233,
#123234,#123235,#123236,#123237,#123238,#123239,#123240,#123241),
 .UNSPECIFIED.,.F.,.F.,(4,3,3,3,3,3,3,3,3,3,3,3,3,3,3,3,3,3,3,3,3,3,3,3,
3,3,3,3,4),(0.,0.0222914007901619,0.045467435982572,0.0675550870544155,
0.0821513218453204,0.0865889302954898,0.110629677084234,0.134994651838372,
0.15933803071403,0.165672897048461,0.170323195429502,0.173916040779313,
0.19899329834446,0.224022472738044,0.248477215576034,0.258554636508914,
0.264135020109551,0.288903368301885,0.314991208014035,0.341079047726185,
0.351267085960766,0.355315309607254,0.381664711215564,0.4034875747766,0.410694463232085,
0.416463282945419,0.443066538202942,0.469275862304378,0.472065635791059),
 .UNSPECIFIED.);
#1142=B_SPLINE_CURVE_WITH_KNOTS('',3,(#123954,#123955,#123956,#123957,#123958,
#123959,#123960,#123961,#123962,#123963,#123964,#123965,#123966,#123967,
#123968,#123969,#123970,#123971,#123972,#123973,#123974,#123975,#123976,
#123977,#123978,#123979,#123980,#123981,#123982,#123983,#123984,#123985,
#123986,#123987,#123988,#123989,#123990,#123991,#123992,#123993,#123994,
#123995,#123996,#123997,#123998,#123999,#124000,#124001,#124002,#124003,
#124004,#124005,#124006,#124007,#124008,#124009,#124010,#124011,#124012,
#124013,#124014,#124015,#124016,#124017,#124018,#124019,#124020,#124021,
#124022,#124023,#124024,#124025,#124026,#124027,#124028,#124029,#124030,
#124031,#124032,#124033,#124034,#124035,#124036,#124037,#124038,#124039,
#124040,#124041),.UNSPECIFIED.,.F.,.F.,(4,3,3,3,3,3,3,3,3,3,3,3,3,3,3,3,
3,3,3,3,3,3,3,3,3,3,3,3,3,4),(7.97682625883415E-15,0.0260517932991782,0.052722550215245,
0.077679095575174,0.0889728027275484,0.0959464342222353,0.10084592545247,
0.1268552016093,0.152534125301528,0.176212517229938,0.186122361708183,0.19254795046146,
0.196620307684512,0.221672220285089,0.246724132885667,0.272050620894862,
0.282513655479386,0.286631738114849,0.31115477174714,0.335765993045936,
0.360166883426141,0.370324928797177,0.375577976589965,0.399326631291423,
0.417608624155145,0.423111148097321,0.427811296634432,0.450556486039327,
0.47164802816752,0.474022601254815),.UNSPECIFIED.);
#2121=SHAPE_REPRESENTATION_RELATIONSHIP('SRR','None',#215646,#2130);
#2130=ADVANCED_BREP_SHAPE_REPRESENTATION('',(#2148),#215602);
#2139=STYLED_ITEM('',(#215698),#2148);
#2148=MANIFOLD_SOLID_BREP('Body1',#28082);
#2173=CYLINDRICAL_SURFACE('',#28273,5.099);
#2174=CYLINDRICAL_SURFACE('',#28275,5.099);
#2175=CYLINDRICAL_SURFACE('',#28276,5.099);
#2176=CYLINDRICAL_SURFACE('',#28277,5.099);
#2177=CYLINDRICAL_SURFACE('',#28279,5.099);
#2178=CYLINDRICAL_SURFACE('',#28281,5.099);
#2179=CYLINDRICAL_SURFACE('',#28282,5.099);
#2180=CYLINDRICAL_SURFACE('',#28283,5.099);
#2181=CYLINDRICAL_SURFACE('',#28285,2.55999999999999);
#2182=CYLINDRICAL_SURFACE('',#28287,2.55999999999999);
#2183=CYLINDRICAL_SURFACE('',#28288,2.55999999999999);
#2184=CYLINDRICAL_SURFACE('',#28289,2.55999999999999);
#2185=CYLINDRICAL_SURFACE('',#28290,2.55999999999999);
#2186=CYLINDRICAL_SURFACE('',#28291,2.55999999999999);
#2187=CYLINDRICAL_SURFACE('',#28292,2.55999999999999);
#2188=CYLINDRICAL_SURFACE('',#28293,2.55999999999999);
#2189=CYLINDRICAL_SURFACE('',#28294,2.55999999999999);
#2190=CYLINDRICAL_SURFACE('',#28295,2.55999999999999);
#2191=CYLINDRICAL_SURFACE('',#28296,2.55999999999999);
#2192=CYLINDRICAL_SURFACE('',#28297,2.55999999999999);
#2193=CYLINDRICAL_SURFACE('',#28298,2.55999999999999);
#2194=CYLINDRICAL_SURFACE('',#28299,2.55999999999999);
#2195=CYLINDRICAL_SURFACE('',#28300,2.55999999999999);
#2196=CYLINDRICAL_SURFACE('',#28301,2.55999999999999);
#2197=CYLINDRICAL_SURFACE('',#28302,2.55999999999999);
#2198=CYLINDRICAL_SURFACE('',#28303,2.55999999999999);
#2199=CYLINDRICAL_SURFACE('',#28304,2.55999999999999);
#2200=CYLINDRICAL_SURFACE('',#28305,2.55999999999999);
#2201=CYLINDRICAL_SURFACE('',#28306,2.55999999999999);
#2202=CYLINDRICAL_SURFACE('',#28307,2.55999999999999);
#2203=CYLINDRICAL_SURFACE('',#28308,2.55999999999999);
#2204=CYLINDRICAL_SURFACE('',#28309,2.55999999999999);
#2205=CYLINDRICAL_SURFACE('',#28310,2.55999999999999);
#2206=CYLINDRICAL_SURFACE('',#28311,2.55999999999999);
#2207=CYLINDRICAL_SURFACE('',#28312,2.55999999999999);
#2208=CYLINDRICAL_SURFACE('',#28314,2.56);
#2209=CYLINDRICAL_SURFACE('',#28316,2.56);
#2210=CYLINDRICAL_SURFACE('',#28317,2.56);
#2211=CYLINDRICAL_SURFACE('',#28318,2.56);
#2212=CYLINDRICAL_SURFACE('',#28319,2.56);
#2213=CYLINDRICAL_SURFACE('',#28320,2.56);
#2214=CYLINDRICAL_SURFACE('',#28321,2.56);
#2215=CYLINDRICAL_SURFACE('',#28322,2.56);
#2216=CYLINDRICAL_SURFACE('',#28323,2.56);
#2217=CYLINDRICAL_SURFACE('',#28324,2.56);
#2218=CYLINDRICAL_SURFACE('',#28325,2.56);
#2219=CYLINDRICAL_SURFACE('',#28326,2.56);
#2220=CYLINDRICAL_SURFACE('',#28327,2.56);
#2221=CYLINDRICAL_SURFACE('',#28328,2.56);
#2222=CYLINDRICAL_SURFACE('',#28329,2.56);
#2223=CYLINDRICAL_SURFACE('',#28330,2.56);
#2224=CYLINDRICAL_SURFACE('',#28331,2.56);
#2225=CYLINDRICAL_SURFACE('',#28332,2.56);
#2226=CYLINDRICAL_SURFACE('',#28333,2.56);
#2227=CYLINDRICAL_SURFACE('',#28334,2.56);
#2228=CYLINDRICAL_SURFACE('',#28335,2.56);
#2229=CYLINDRICAL_SURFACE('',#28336,2.56);
#2230=CYLINDRICAL_SURFACE('',#28337,2.56);
#2231=CYLINDRICAL_SURFACE('',#28338,2.56);
#2232=CYLINDRICAL_SURFACE('',#28339,2.56);
#2233=CYLINDRICAL_SURFACE('',#28340,2.56);
#2234=CYLINDRICAL_SURFACE('',#28341,2.56);
#2235=CYLINDRICAL_SURFACE('',#28343,2.56);
#2236=CYLINDRICAL_SURFACE('',#28345,2.56);
#2237=CYLINDRICAL_SURFACE('',#28346,2.56);
#2238=CYLINDRICAL_SURFACE('',#28347,2.56);
#2239=CYLINDRICAL_SURFACE('',#28348,2.56);
#2240=CYLINDRICAL_SURFACE('',#28349,2.56);
#2241=CYLINDRICAL_SURFACE('',#28350,2.56);
#2242=CYLINDRICAL_SURFACE('',#28351,2.56);
#2243=CYLINDRICAL_SURFACE('',#28352,2.56);
#2244=CYLINDRICAL_SURFACE('',#28353,2.56);
#2245=CYLINDRICAL_SURFACE('',#28354,2.56);
#2246=CYLINDRICAL_SURFACE('',#28355,2.56);
#2247=CYLINDRICAL_SURFACE('',#28356,2.56);
#2248=CYLINDRICAL_SURFACE('',#28357,2.56);
#2249=CYLINDRICAL_SURFACE('',#28358,2.56);
#2250=CYLINDRICAL_SURFACE('',#28359,2.56);
#2251=CYLINDRICAL_SURFACE('',#28360,2.56);
#2252=CYLINDRICAL_SURFACE('',#28361,2.56);
#2253=CYLINDRICAL_SURFACE('',#28362,2.56);
#2254=CYLINDRICAL_SURFACE('',#28363,2.56);
#2255=CYLINDRICAL_SURFACE('',#28364,2.56);
#2256=CYLINDRICAL_SURFACE('',#28365,2.56);
#2257=CYLINDRICAL_SURFACE('',#28366,2.56);
#2258=CYLINDRICAL_SURFACE('',#28367,2.56);
#2259=CYLINDRICAL_SURFACE('',#28368,2.56);
#2260=CYLINDRICAL_SURFACE('',#28369,2.56);
#2261=CYLINDRICAL_SURFACE('',#28370,2.56);
#2262=CYLINDRICAL_SURFACE('',#28372,2.56);
#2263=CYLINDRICAL_SURFACE('',#28374,2.56);
#2264=CYLINDRICAL_SURFACE('',#28375,2.56);
#2265=CYLINDRICAL_SURFACE('',#28376,2.56);
#2266=CYLINDRICAL_SURFACE('',#28377,2.56);
#2267=CYLINDRICAL_SURFACE('',#28378,2.56);
#2268=CYLINDRICAL_SURFACE('',#28379,2.56);
#2269=CYLINDRICAL_SURFACE('',#28380,2.56);
#2270=CYLINDRICAL_SURFACE('',#28381,2.56);
#2271=CYLINDRICAL_SURFACE('',#28382,2.56);
#2272=CYLINDRICAL_SURFACE('',#28383,2.56);
#2273=CYLINDRICAL_SURFACE('',#28384,2.56);
#2274=CYLINDRICAL_SURFACE('',#28385,2.56);
#2275=CYLINDRICAL_SURFACE('',#28386,2.56);
#2276=CYLINDRICAL_SURFACE('',#28387,2.56);
#2277=CYLINDRICAL_SURFACE('',#28388,2.56);
#2278=CYLINDRICAL_SURFACE('',#28389,2.56);
#2279=CYLINDRICAL_SURFACE('',#28390,2.56);
#2280=CYLINDRICAL_SURFACE('',#28391,2.56);
#2281=CYLINDRICAL_SURFACE('',#28392,2.56);
#2282=CYLINDRICAL_SURFACE('',#28393,2.56);
#2283=CYLINDRICAL_SURFACE('',#28394,2.56);
#2284=CYLINDRICAL_SURFACE('',#28395,2.56);
#2285=CYLINDRICAL_SURFACE('',#28396,2.56);
#2286=CYLINDRICAL_SURFACE('',#28397,2.56);
#2287=CYLINDRICAL_SURFACE('',#28398,2.56);
#2288=CYLINDRICAL_SURFACE('',#28399,2.56);
#2289=CYLINDRICAL_SURFACE('',#28401,4.263);
#2290=CYLINDRICAL_SURFACE('',#28403,4.263);
#2291=CYLINDRICAL_SURFACE('',#28404,4.263);
#2292=CYLINDRICAL_SURFACE('',#28405,4.263);
#2293=CYLINDRICAL_SURFACE('',#28407,4.263);
#2294=CYLINDRICAL_SURFACE('',#28409,4.263);
#2295=CYLINDRICAL_SURFACE('',#28411,4.263);
#2296=CYLINDRICAL_SURFACE('',#28412,4.263);
#2297=CYLINDRICAL_SURFACE('',#28414,2.117);
#2298=CYLINDRICAL_SURFACE('',#28416,2.117);
#2299=CYLINDRICAL_SURFACE('',#28417,2.117);
#2300=CYLINDRICAL_SURFACE('',#28418,2.117);
#2301=CYLINDRICAL_SURFACE('',#28419,2.117);
#2302=CYLINDRICAL_SURFACE('',#28420,2.117);
#2303=CYLINDRICAL_SURFACE('',#28421,2.117);
#2304=CYLINDRICAL_SURFACE('',#28422,2.117);
#2305=CYLINDRICAL_SURFACE('',#28423,2.117);
#2306=CYLINDRICAL_SURFACE('',#28424,2.117);
#2307=CYLINDRICAL_SURFACE('',#28425,2.117);
#2308=CYLINDRICAL_SURFACE('',#28426,2.117);
#2309=CYLINDRICAL_SURFACE('',#28427,2.117);
#2310=CYLINDRICAL_SURFACE('',#28428,2.117);
#2311=CYLINDRICAL_SURFACE('',#28429,2.117);
#2312=CYLINDRICAL_SURFACE('',#28430,2.117);
#2313=CYLINDRICAL_SURFACE('',#28431,2.117);
#2314=CYLINDRICAL_SURFACE('',#28432,2.117);
#2315=CYLINDRICAL_SURFACE('',#28433,2.117);
#2316=CYLINDRICAL_SURFACE('',#28434,2.117);
#2317=CYLINDRICAL_SURFACE('',#28435,2.117);
#2318=CYLINDRICAL_SURFACE('',#28436,2.117);
#2319=CYLINDRICAL_SURFACE('',#28437,2.117);
#2320=CYLINDRICAL_SURFACE('',#28438,2.117);
#2321=CYLINDRICAL_SURFACE('',#28439,2.117);
#2322=CYLINDRICAL_SURFACE('',#28440,2.117);
#2323=CYLINDRICAL_SURFACE('',#28441,2.117);
#2324=CYLINDRICAL_SURFACE('',#28443,2.117);
#2325=CYLINDRICAL_SURFACE('',#28445,2.117);
#2326=CYLINDRICAL_SURFACE('',#28446,2.117);
#2327=CYLINDRICAL_SURFACE('',#28447,2.117);
#2328=CYLINDRICAL_SURFACE('',#28448,2.117);
#2329=CYLINDRICAL_SURFACE('',#28449,2.117);
#2330=CYLINDRICAL_SURFACE('',#28450,2.117);
#2331=CYLINDRICAL_SURFACE('',#28451,2.117);
#2332=CYLINDRICAL_SURFACE('',#28452,2.117);
#2333=CYLINDRICAL_SURFACE('',#28453,2.117);
#2334=CYLINDRICAL_SURFACE('',#28454,2.117);
#2335=CYLINDRICAL_SURFACE('',#28455,2.117);
#2336=CYLINDRICAL_SURFACE('',#28456,2.117);
#2337=CYLINDRICAL_SURFACE('',#28457,2.117);
#2338=CYLINDRICAL_SURFACE('',#28458,2.117);
#2339=CYLINDRICAL_SURFACE('',#28459,2.117);
#2340=CYLINDRICAL_SURFACE('',#28460,2.117);
#2341=CYLINDRICAL_SURFACE('',#28461,2.117);
#2342=CYLINDRICAL_SURFACE('',#28462,2.117);
#2343=CYLINDRICAL_SURFACE('',#28463,2.117);
#2344=CYLINDRICAL_SURFACE('',#28464,2.117);
#2345=CYLINDRICAL_SURFACE('',#28465,2.117);
#2346=CYLINDRICAL_SURFACE('',#28466,2.117);
#2347=CYLINDRICAL_SURFACE('',#28467,2.117);
#2348=CYLINDRICAL_SURFACE('',#28468,2.117);
#2349=CYLINDRICAL_SURFACE('',#28469,2.117);
#2350=CYLINDRICAL_SURFACE('',#28470,2.117);
#2351=CYLINDRICAL_SURFACE('',#28472,2.117);
#2352=CYLINDRICAL_SURFACE('',#28474,2.117);
#2353=CYLINDRICAL_SURFACE('',#28475,2.117);
#2354=CYLINDRICAL_SURFACE('',#28476,2.117);
#2355=CYLINDRICAL_SURFACE('',#28477,2.117);
#2356=CYLINDRICAL_SURFACE('',#28478,2.117);
#2357=CYLINDRICAL_SURFACE('',#28479,2.117);
#2358=CYLINDRICAL_SURFACE('',#28480,2.117);
#2359=CYLINDRICAL_SURFACE('',#28481,2.117);
#2360=CYLINDRICAL_SURFACE('',#28482,2.117);
#2361=CYLINDRICAL_SURFACE('',#28483,2.117);
#2362=CYLINDRICAL_SURFACE('',#28484,2.117);
#2363=CYLINDRICAL_SURFACE('',#28485,2.117);
#2364=CYLINDRICAL_SURFACE('',#28486,2.117);
#2365=CYLINDRICAL_SURFACE('',#28487,2.117);
#2366=CYLINDRICAL_SURFACE('',#28488,2.117);
#2367=CYLINDRICAL_SURFACE('',#28489,2.117);
#2368=CYLINDRICAL_SURFACE('',#28490,2.117);
#2369=CYLINDRICAL_SURFACE('',#28491,2.117);
#2370=CYLINDRICAL_SURFACE('',#28492,2.117);
#2371=CYLINDRICAL_SURFACE('',#28493,2.117);
#2372=CYLINDRICAL_SURFACE('',#28494,2.117);
#2373=CYLINDRICAL_SURFACE('',#28495,2.117);
#2374=CYLINDRICAL_SURFACE('',#28496,2.117);
#2375=CYLINDRICAL_SURFACE('',#28497,2.117);
#2376=CYLINDRICAL_SURFACE('',#28498,2.117);
#2377=CYLINDRICAL_SURFACE('',#28499,2.117);
#2378=CYLINDRICAL_SURFACE('',#28501,2.117);
#2379=CYLINDRICAL_SURFACE('',#28503,2.117);
#2380=CYLINDRICAL_SURFACE('',#28504,2.117);
#2381=CYLINDRICAL_SURFACE('',#28505,2.117);
#2382=CYLINDRICAL_SURFACE('',#28506,2.117);
#2383=CYLINDRICAL_SURFACE('',#28507,2.117);
#2384=CYLINDRICAL_SURFACE('',#28508,2.117);
#2385=CYLINDRICAL_SURFACE('',#28509,2.117);
#2386=CYLINDRICAL_SURFACE('',#28510,2.117);
#2387=CYLINDRICAL_SURFACE('',#28511,2.117);
#2388=CYLINDRICAL_SURFACE('',#28512,2.117);
#2389=CYLINDRICAL_SURFACE('',#28513,2.117);
#2390=CYLINDRICAL_SURFACE('',#28514,2.117);
#2391=CYLINDRICAL_SURFACE('',#28515,2.117);
#2392=CYLINDRICAL_SURFACE('',#28516,2.117);
#2393=CYLINDRICAL_SURFACE('',#28517,2.117);
#2394=CYLINDRICAL_SURFACE('',#28518,2.117);
#2395=CYLINDRICAL_SURFACE('',#28519,2.117);
#2396=CYLINDRICAL_SURFACE('',#28520,2.117);
#2397=CYLINDRICAL_SURFACE('',#28521,2.117);
#2398=CYLINDRICAL_SURFACE('',#28522,2.117);
#2399=CYLINDRICAL_SURFACE('',#28523,2.117);
#2400=CYLINDRICAL_SURFACE('',#28524,2.117);
#2401=CYLINDRICAL_SURFACE('',#28525,2.117);
#2402=CYLINDRICAL_SURFACE('',#28526,2.117);
#2403=CYLINDRICAL_SURFACE('',#28527,2.117);
#2404=CYLINDRICAL_SURFACE('',#28528,2.117);
#2405=CYLINDRICAL_SURFACE('',#28530,2.117);
#2406=CYLINDRICAL_SURFACE('',#28531,2.117);
#2407=CYLINDRICAL_SURFACE('',#28532,2.117);
#2408=CYLINDRICAL_SURFACE('',#28533,2.117);
#2409=CYLINDRICAL_SURFACE('',#28534,4.263);
#2410=CYLINDRICAL_SURFACE('',#28535,4.263);
#2411=CYLINDRICAL_SURFACE('',#28537,2.56);
#2412=CYLINDRICAL_SURFACE('',#28538,2.56);
#2413=CYLINDRICAL_SURFACE('',#28539,2.56);
#2414=CYLINDRICAL_SURFACE('',#28540,2.55999999999999);
#2415=CYLINDRICAL_SURFACE('',#28541,5.099);
#2416=CYLINDRICAL_SURFACE('',#28542,5.099);
#2417=CYLINDRICAL_SURFACE('',#28543,4.);
#2418=CYLINDRICAL_SURFACE('',#28547,4.5);
#2419=CYLINDRICAL_SURFACE('',#28552,4.);
#2420=CYLINDRICAL_SURFACE('',#28556,4.5);
#2421=CYLINDRICAL_SURFACE('',#28561,5.);
#2422=CYLINDRICAL_SURFACE('',#28588,3.);
#2423=CYLINDRICAL_SURFACE('',#28592,6.);
#2424=CYLINDRICAL_SURFACE('',#28596,6.);
#2425=CYLINDRICAL_SURFACE('',#28611,3.);
#2426=CYLINDRICAL_SURFACE('',#28617,4.);
#2427=CYLINDRICAL_SURFACE('',#28621,5.);
#2428=CYLINDRICAL_SURFACE('',#28624,6.);
#2429=CYLINDRICAL_SURFACE('',#28628,6.);
#2430=CYLINDRICAL_SURFACE('',#28643,3.);
#2431=CYLINDRICAL_SURFACE('',#28654,3.);
#2432=CYLINDRICAL_SURFACE('',#28662,5.);
#2433=CYLINDRICAL_SURFACE('',#28665,4.);
#2434=CYLINDRICAL_SURFACE('',#28668,2.5);
#2435=CYLINDRICAL_SURFACE('',#28671,2.5);
#2436=CYLINDRICAL_SURFACE('',#28675,3.99143708455989);
#2437=CYLINDRICAL_SURFACE('',#28677,0.190999999999999);
#2438=CYLINDRICAL_SURFACE('',#28680,0.190999999999999);
#2439=CYLINDRICAL_SURFACE('',#28683,0.254);
#2440=CYLINDRICAL_SURFACE('',#28686,5.);
#2441=CYLINDRICAL_SURFACE('',#28688,5.);
#2442=CYLINDRICAL_SURFACE('',#28691,5.);
#2443=CYLINDRICAL_SURFACE('',#28694,5.);
#2444=CYLINDRICAL_SURFACE('',#28697,0.253999999999999);
#2445=CYLINDRICAL_SURFACE('',#28700,0.190999999999999);
#2446=CYLINDRICAL_SURFACE('',#28703,0.191);
#2447=CYLINDRICAL_SURFACE('',#28706,3.9914370845599);
#3019=FACE_OUTER_BOUND('',#4332,.T.);
#3020=FACE_OUTER_BOUND('',#4333,.T.);
#3021=FACE_OUTER_BOUND('',#4334,.T.);
#3022=FACE_OUTER_BOUND('',#4335,.T.);
#3023=FACE_OUTER_BOUND('',#4336,.T.);
#3024=FACE_OUTER_BOUND('',#4337,.T.);
#3025=FACE_OUTER_BOUND('',#4338,.T.);
#3026=FACE_OUTER_BOUND('',#4339,.T.);
#3027=FACE_OUTER_BOUND('',#4340,.T.);
#3028=FACE_OUTER_BOUND('',#4341,.T.);
#3029=FACE_OUTER_BOUND('',#4342,.T.);
#3030=FACE_OUTER_BOUND('',#4343,.T.);
#3031=FACE_OUTER_BOUND('',#4344,.T.);
#3032=FACE_OUTER_BOUND('',#4345,.T.);
#3033=FACE_OUTER_BOUND('',#4346,.T.);
#3034=FACE_OUTER_BOUND('',#4347,.T.);
#3035=FACE_OUTER_BOUND('',#4348,.T.);
#3036=FACE_OUTER_BOUND('',#4349,.T.);
#3037=FACE_OUTER_BOUND('',#4350,.T.);
#3038=FACE_OUTER_BOUND('',#4351,.T.);
#3039=FACE_OUTER_BOUND('',#4352,.T.);
#3040=FACE_OUTER_BOUND('',#4353,.T.);
#3041=FACE_OUTER_BOUND('',#4354,.T.);
#3042=FACE_OUTER_BOUND('',#4355,.T.);
#3043=FACE_OUTER_BOUND('',#4356,.T.);
#3044=FACE_OUTER_BOUND('',#4357,.T.);
#3045=FACE_OUTER_BOUND('',#4358,.T.);
#3046=FACE_OUTER_BOUND('',#4359,.T.);
#3047=FACE_OUTER_BOUND('',#4360,.T.);
#3048=FACE_OUTER_BOUND('',#4361,.T.);
#3049=FACE_OUTER_BOUND('',#4362,.T.);
#3050=FACE_OUTER_BOUND('',#4363,.T.);
#3051=FACE_OUTER_BOUND('',#4364,.T.);
#3052=FACE_OUTER_BOUND('',#4365,.T.);
#3053=FACE_OUTER_BOUND('',#4366,.T.);
#3054=FACE_OUTER_BOUND('',#4367,.T.);
#3055=FACE_OUTER_BOUND('',#4368,.T.);
#3056=FACE_OUTER_BOUND('',#4369,.T.);
#3057=FACE_OUTER_BOUND('',#4370,.T.);
#3058=FACE_OUTER_BOUND('',#4371,.T.);
#3059=FACE_OUTER_BOUND('',#4372,.T.);
#3060=FACE_OUTER_BOUND('',#4373,.T.);
#3061=FACE_OUTER_BOUND('',#4374,.T.);
#3062=FACE_OUTER_BOUND('',#4375,.T.);
#3063=FACE_OUTER_BOUND('',#4376,.T.);
#3064=FACE_OUTER_BOUND('',#4377,.T.);
#3065=FACE_OUTER_BOUND('',#4378,.T.);
#3066=FACE_OUTER_BOUND('',#4379,.T.);
#3067=FACE_OUTER_BOUND('',#4380,.T.);
#3068=FACE_OUTER_BOUND('',#4381,.T.);
#3069=FACE_OUTER_BOUND('',#4382,.T.);
#3070=FACE_OUTER_BOUND('',#4383,.T.);
#3071=FACE_OUTER_BOUND('',#4384,.T.);
#3072=FACE_OUTER_BOUND('',#4385,.T.);
#3073=FACE_OUTER_BOUND('',#4386,.T.);
#3074=FACE_OUTER_BOUND('',#4387,.T.);
#3075=FACE_OUTER_BOUND('',#4388,.T.);
#3076=FACE_OUTER_BOUND('',#4389,.T.);
#3077=FACE_OUTER_BOUND('',#4390,.T.);
#3078=FACE_OUTER_BOUND('',#4391,.T.);
#3079=FACE_OUTER_BOUND('',#4392,.T.);
#3080=FACE_OUTER_BOUND('',#4393,.T.);
#3081=FACE_OUTER_BOUND('',#4394,.T.);
#3082=FACE_OUTER_BOUND('',#4395,.T.);
#3083=FACE_OUTER_BOUND('',#4396,.T.);
#3084=FACE_OUTER_BOUND('',#4397,.T.);
#3085=FACE_OUTER_BOUND('',#4398,.T.);
#3086=FACE_OUTER_BOUND('',#4399,.T.);
#3087=FACE_OUTER_BOUND('',#4400,.T.);
#3088=FACE_OUTER_BOUND('',#4401,.T.);
#3089=FACE_OUTER_BOUND('',#4402,.T.);
#3090=FACE_OUTER_BOUND('',#4403,.T.);
#3091=FACE_OUTER_BOUND('',#4404,.T.);
#3092=FACE_OUTER_BOUND('',#4405,.T.);
#3093=FACE_OUTER_BOUND('',#4406,.T.);
#3094=FACE_OUTER_BOUND('',#4407,.T.);
#3095=FACE_OUTER_BOUND('',#4408,.T.);
#3096=FACE_OUTER_BOUND('',#4409,.T.);
#3097=FACE_OUTER_BOUND('',#4410,.T.);
#3098=FACE_OUTER_BOUND('',#4411,.T.);
#3099=FACE_OUTER_BOUND('',#4412,.T.);
#3100=FACE_OUTER_BOUND('',#4413,.T.);
#3101=FACE_OUTER_BOUND('',#4414,.T.);
#3102=FACE_OUTER_BOUND('',#4415,.T.);
#3103=FACE_OUTER_BOUND('',#4416,.T.);
#3104=FACE_OUTER_BOUND('',#4417,.T.);
#3105=FACE_OUTER_BOUND('',#4418,.T.);
#3106=FACE_OUTER_BOUND('',#4419,.T.);
#3107=FACE_OUTER_BOUND('',#4420,.T.);
#3108=FACE_OUTER_BOUND('',#4421,.T.);
#3109=FACE_OUTER_BOUND('',#4422,.T.);
#3110=FACE_OUTER_BOUND('',#4423,.T.);
#3111=FACE_OUTER_BOUND('',#4424,.T.);
#3112=FACE_OUTER_BOUND('',#4425,.T.);
#3113=FACE_OUTER_BOUND('',#4426,.T.);
#3114=FACE_OUTER_BOUND('',#4427,.T.);
#3115=FACE_OUTER_BOUND('',#4428,.T.);
#3116=FACE_OUTER_BOUND('',#4429,.T.);
#3117=FACE_OUTER_BOUND('',#4430,.T.);
#3118=FACE_OUTER_BOUND('',#4431,.T.);
#3119=FACE_OUTER_BOUND('',#4432,.T.);
#3120=FACE_OUTER_BOUND('',#4433,.T.);
#3121=FACE_OUTER_BOUND('',#4434,.T.);
#3122=FACE_OUTER_BOUND('',#4435,.T.);
#3123=FACE_OUTER_BOUND('',#4436,.T.);
#3124=FACE_OUTER_BOUND('',#4437,.T.);
#3125=FACE_OUTER_BOUND('',#4438,.T.);
#3126=FACE_OUTER_BOUND('',#4439,.T.);
#3127=FACE_OUTER_BOUND('',#4440,.T.);
#3128=FACE_OUTER_BOUND('',#4441,.T.);
#3129=FACE_OUTER_BOUND('',#4442,.T.);
#3130=FACE_OUTER_BOUND('',#4443,.T.);
#3131=FACE_OUTER_BOUND('',#4444,.T.);
#3132=FACE_OUTER_BOUND('',#4445,.T.);
#3133=FACE_OUTER_BOUND('',#4446,.T.);
#3134=FACE_OUTER_BOUND('',#4447,.T.);
#3135=FACE_OUTER_BOUND('',#4448,.T.);
#3136=FACE_OUTER_BOUND('',#4449,.T.);
#3137=FACE_OUTER_BOUND('',#4450,.T.);
#3138=FACE_OUTER_BOUND('',#4451,.T.);
#3139=FACE_OUTER_BOUND('',#4452,.T.);
#3140=FACE_OUTER_BOUND('',#4453,.T.);
#3141=FACE_OUTER_BOUND('',#4454,.T.);
#3142=FACE_OUTER_BOUND('',#4455,.T.);
#3143=FACE_OUTER_BOUND('',#4456,.T.);
#3144=FACE_OUTER_BOUND('',#4457,.T.);
#3145=FACE_OUTER_BOUND('',#4458,.T.);
#3146=FACE_OUTER_BOUND('',#4459,.T.);
#3147=FACE_OUTER_BOUND('',#4460,.T.);
#3148=FACE_OUTER_BOUND('',#4461,.T.);
#3149=FACE_OUTER_BOUND('',#4462,.T.);
#3150=FACE_OUTER_BOUND('',#4463,.T.);
#3151=FACE_OUTER_BOUND('',#4464,.T.);
#3152=FACE_OUTER_BOUND('',#4465,.T.);
#3153=FACE_OUTER_BOUND('',#4466,.T.);
#3154=FACE_OUTER_BOUND('',#4467,.T.);
#3155=FACE_OUTER_BOUND('',#4468,.T.);
#3156=FACE_OUTER_BOUND('',#4469,.T.);
#3157=FACE_OUTER_BOUND('',#4470,.T.);
#3158=FACE_OUTER_BOUND('',#4471,.T.);
#3159=FACE_OUTER_BOUND('',#4472,.T.);
#3160=FACE_OUTER_BOUND('',#4473,.T.);
#3161=FACE_OUTER_BOUND('',#4474,.T.);
#3162=FACE_OUTER_BOUND('',#4475,.T.);
#3163=FACE_OUTER_BOUND('',#4476,.T.);
#3164=FACE_OUTER_BOUND('',#4477,.T.);
#3165=FACE_OUTER_BOUND('',#4478,.T.);
#3166=FACE_OUTER_BOUND('',#4479,.T.);
#3167=FACE_OUTER_BOUND('',#4480,.T.);
#3168=FACE_OUTER_BOUND('',#4481,.T.);
#3169=FACE_OUTER_BOUND('',#4482,.T.);
#3170=FACE_OUTER_BOUND('',#4483,.T.);
#3171=FACE_OUTER_BOUND('',#4484,.T.);
#3172=FACE_OUTER_BOUND('',#4485,.T.);
#3173=FACE_OUTER_BOUND('',#4486,.T.);
#3174=FACE_OUTER_BOUND('',#4487,.T.);
#3175=FACE_OUTER_BOUND('',#4488,.T.);
#3176=FACE_OUTER_BOUND('',#4489,.T.);
#3177=FACE_OUTER_BOUND('',#4490,.T.);
#3178=FACE_OUTER_BOUND('',#4491,.T.);
#3179=FACE_OUTER_BOUND('',#4492,.T.);
#3180=FACE_OUTER_BOUND('',#4493,.T.);
#3181=FACE_OUTER_BOUND('',#4494,.T.);
#3182=FACE_OUTER_BOUND('',#4495,.T.);
#3183=FACE_OUTER_BOUND('',#4496,.T.);
#3184=FACE_OUTER_BOUND('',#4497,.T.);
#3185=FACE_OUTER_BOUND('',#4498,.T.);
#3186=FACE_OUTER_BOUND('',#4499,.T.);
#3187=FACE_OUTER_BOUND('',#4500,.T.);
#3188=FACE_OUTER_BOUND('',#4501,.T.);
#3189=FACE_OUTER_BOUND('',#4502,.T.);
#3190=FACE_OUTER_BOUND('',#4503,.T.);
#3191=FACE_OUTER_BOUND('',#4504,.T.);
#3192=FACE_OUTER_BOUND('',#4505,.T.);
#3193=FACE_OUTER_BOUND('',#4506,.T.);
#3194=FACE_OUTER_BOUND('',#4507,.T.);
#3195=FACE_OUTER_BOUND('',#4508,.T.);
#3196=FACE_OUTER_BOUND('',#4509,.T.);
#3197=FACE_OUTER_BOUND('',#4510,.T.);
#3198=FACE_OUTER_BOUND('',#4511,.T.);
#3199=FACE_OUTER_BOUND('',#4512,.T.);
#3200=FACE_OUTER_BOUND('',#4513,.T.);
#3201=FACE_OUTER_BOUND('',#4514,.T.);
#3202=FACE_OUTER_BOUND('',#4515,.T.);
#3203=FACE_OUTER_BOUND('',#4516,.T.);
#3204=FACE_OUTER_BOUND('',#4517,.T.);
#3205=FACE_OUTER_BOUND('',#4518,.T.);
#3206=FACE_OUTER_BOUND('',#4519,.T.);
#3207=FACE_OUTER_BOUND('',#4520,.T.);
#3208=FACE_OUTER_BOUND('',#4521,.T.);
#3209=FACE_OUTER_BOUND('',#4522,.T.);
#3210=FACE_OUTER_BOUND('',#4523,.T.);
#3211=FACE_OUTER_BOUND('',#4524,.T.);
#3212=FACE_OUTER_BOUND('',#4525,.T.);
#3213=FACE_OUTER_BOUND('',#4526,.T.);
#3214=FACE_OUTER_BOUND('',#4527,.T.);
#3215=FACE_OUTER_BOUND('',#4528,.T.);
#3216=FACE_OUTER_BOUND('',#4529,.T.);
#3217=FACE_OUTER_BOUND('',#4530,.T.);
#3218=FACE_OUTER_BOUND('',#4531,.T.);
#3219=FACE_OUTER_BOUND('',#4532,.T.);
#3220=FACE_OUTER_BOUND('',#4533,.T.);
#3221=FACE_OUTER_BOUND('',#4534,.T.);
#3222=FACE_OUTER_BOUND('',#4535,.T.);
#3223=FACE_OUTER_BOUND('',#4536,.T.);
#3224=FACE_OUTER_BOUND('',#4537,.T.);
#3225=FACE_OUTER_BOUND('',#4538,.T.);
#3226=FACE_OUTER_BOUND('',#4539,.T.);
#3227=FACE_OUTER_BOUND('',#4540,.T.);
#3228=FACE_OUTER_BOUND('',#4541,.T.);
#3229=FACE_OUTER_BOUND('',#4542,.T.);
#3230=FACE_OUTER_BOUND('',#4543,.T.);
#3231=FACE_OUTER_BOUND('',#4544,.T.);
#3232=FACE_OUTER_BOUND('',#4545,.T.);
#3233=FACE_OUTER_BOUND('',#4546,.T.);
#3234=FACE_OUTER_BOUND('',#4547,.T.);
#3235=FACE_OUTER_BOUND('',#4548,.T.);
#3236=FACE_OUTER_BOUND('',#4549,.T.);
#3237=FACE_OUTER_BOUND('',#4550,.T.);
#3238=FACE_OUTER_BOUND('',#4551,.T.);
#3239=FACE_OUTER_BOUND('',#4552,.T.);
#3240=FACE_OUTER_BOUND('',#4553,.T.);
#3241=FACE_OUTER_BOUND('',#4554,.T.);
#3242=FACE_OUTER_BOUND('',#4555,.T.);
#3243=FACE_OUTER_BOUND('',#4556,.T.);
#3244=FACE_OUTER_BOUND('',#4557,.T.);
#3245=FACE_OUTER_BOUND('',#4558,.T.);
#3246=FACE_OUTER_BOUND('',#4559,.T.);
#3247=FACE_OUTER_BOUND('',#4560,.T.);
#3248=FACE_OUTER_BOUND('',#4561,.T.);
#3249=FACE_OUTER_BOUND('',#4562,.T.);
#3250=FACE_OUTER_BOUND('',#4563,.T.);
#3251=FACE_OUTER_BOUND('',#4564,.T.);
#3252=FACE_OUTER_BOUND('',#4565,.T.);
#3253=FACE_OUTER_BOUND('',#4566,.T.);
#3254=FACE_OUTER_BOUND('',#4567,.T.);
#3255=FACE_OUTER_BOUND('',#4568,.T.);
#3256=FACE_OUTER_BOUND('',#4569,.T.);
#3257=FACE_OUTER_BOUND('',#4570,.T.);
#3258=FACE_OUTER_BOUND('',#4571,.T.);
#3259=FACE_OUTER_BOUND('',#4572,.T.);
#3260=FACE_OUTER_BOUND('',#4573,.T.);
#3261=FACE_OUTER_BOUND('',#4574,.T.);
#3262=FACE_OUTER_BOUND('',#4575,.T.);
#3263=FACE_OUTER_BOUND('',#4576,.T.);
#3264=FACE_OUTER_BOUND('',#4577,.T.);
#3265=FACE_OUTER_BOUND('',#4578,.T.);
#3266=FACE_OUTER_BOUND('',#4579,.T.);
#3267=FACE_OUTER_BOUND('',#4580,.T.);
#3268=FACE_OUTER_BOUND('',#4581,.T.);
#3269=FACE_OUTER_BOUND('',#4582,.T.);
#3270=FACE_OUTER_BOUND('',#4583,.T.);
#3271=FACE_OUTER_BOUND('',#4584,.T.);
#3272=FACE_OUTER_BOUND('',#4585,.T.);
#3273=FACE_OUTER_BOUND('',#4586,.T.);
#3274=FACE_OUTER_BOUND('',#4587,.T.);
#3275=FACE_OUTER_BOUND('',#4588,.T.);
#3276=FACE_OUTER_BOUND('',#4589,.T.);
#3277=FACE_OUTER_BOUND('',#4599,.T.);
#3278=FACE_OUTER_BOUND('',#4600,.T.);
#3279=FACE_OUTER_BOUND('',#4601,.T.);
#3280=FACE_OUTER_BOUND('',#4602,.T.);
#3281=FACE_OUTER_BOUND('',#4603,.T.);
#3282=FACE_OUTER_BOUND('',#4604,.T.);
#3283=FACE_OUTER_BOUND('',#4605,.T.);
#3284=FACE_OUTER_BOUND('',#4606,.T.);
#3285=FACE_OUTER_BOUND('',#4607,.T.);
#3286=FACE_OUTER_BOUND('',#4608,.T.);
#3287=FACE_OUTER_BOUND('',#4609,.T.);
#3288=FACE_OUTER_BOUND('',#4610,.T.);
#3289=FACE_OUTER_BOUND('',#4611,.T.);
#3290=FACE_OUTER_BOUND('',#4612,.T.);
#3291=FACE_OUTER_BOUND('',#4613,.T.);
#3292=FACE_OUTER_BOUND('',#4614,.T.);
#3293=FACE_OUTER_BOUND('',#4615,.T.);
#3294=FACE_OUTER_BOUND('',#4616,.T.);
#3295=FACE_OUTER_BOUND('',#4617,.T.);
#3296=FACE_OUTER_BOUND('',#4618,.T.);
#3297=FACE_OUTER_BOUND('',#4619,.T.);
#3298=FACE_OUTER_BOUND('',#4621,.T.);
#3299=FACE_OUTER_BOUND('',#4622,.T.);
#3300=FACE_OUTER_BOUND('',#4623,.T.);
#3301=FACE_OUTER_BOUND('',#4624,.T.);
#3302=FACE_OUTER_BOUND('',#4625,.T.);
#3303=FACE_OUTER_BOUND('',#4626,.T.);
#3304=FACE_OUTER_BOUND('',#4630,.T.);
#3305=FACE_OUTER_BOUND('',#4631,.T.);
#3306=FACE_OUTER_BOUND('',#4632,.T.);
#3307=FACE_OUTER_BOUND('',#4633,.T.);
#3308=FACE_OUTER_BOUND('',#4634,.T.);
#3309=FACE_OUTER_BOUND('',#4635,.T.);
#3310=FACE_OUTER_BOUND('',#4636,.T.);
#3311=FACE_OUTER_BOUND('',#4637,.T.);
#3312=FACE_OUTER_BOUND('',#4638,.T.);
#3313=FACE_OUTER_BOUND('',#4640,.T.);
#3314=FACE_OUTER_BOUND('',#4641,.T.);
#3315=FACE_OUTER_BOUND('',#4642,.T.);
#3316=FACE_OUTER_BOUND('',#4643,.T.);
#3317=FACE_OUTER_BOUND('',#4644,.T.);
#3318=FACE_OUTER_BOUND('',#4645,.T.);
#3319=FACE_OUTER_BOUND('',#4646,.T.);
#3320=FACE_OUTER_BOUND('',#4647,.T.);
#3321=FACE_OUTER_BOUND('',#4648,.T.);
#3322=FACE_OUTER_BOUND('',#4649,.T.);
#3323=FACE_OUTER_BOUND('',#4650,.T.);
#3324=FACE_OUTER_BOUND('',#4651,.T.);
#3325=FACE_OUTER_BOUND('',#4652,.T.);
#3326=FACE_OUTER_BOUND('',#4656,.T.);
#3327=FACE_OUTER_BOUND('',#4657,.T.);
#3328=FACE_OUTER_BOUND('',#4658,.T.);
#3329=FACE_OUTER_BOUND('',#4659,.T.);
#3330=FACE_OUTER_BOUND('',#4660,.T.);
#3331=FACE_OUTER_BOUND('',#4661,.T.);
#3332=FACE_OUTER_BOUND('',#4662,.T.);
#3333=FACE_OUTER_BOUND('',#4663,.T.);
#3334=FACE_OUTER_BOUND('',#4664,.T.);
#3335=FACE_OUTER_BOUND('',#4666,.T.);
#3336=FACE_OUTER_BOUND('',#4667,.T.);
#3337=FACE_OUTER_BOUND('',#4668,.T.);
#3338=FACE_OUTER_BOUND('',#4669,.T.);
#3339=FACE_OUTER_BOUND('',#4670,.T.);
#3340=FACE_OUTER_BOUND('',#4671,.T.);
#3341=FACE_OUTER_BOUND('',#4672,.T.);
#3342=FACE_OUTER_BOUND('',#4673,.T.);
#3343=FACE_OUTER_BOUND('',#4674,.T.);
#3344=FACE_OUTER_BOUND('',#4676,.T.);
#3345=FACE_OUTER_BOUND('',#4677,.T.);
#3346=FACE_OUTER_BOUND('',#4678,.T.);
#3347=FACE_OUTER_BOUND('',#4681,.T.);
#3348=FACE_OUTER_BOUND('',#4682,.T.);
#3349=FACE_OUTER_BOUND('',#4683,.T.);
#3350=FACE_OUTER_BOUND('',#4684,.T.);
#3351=FACE_OUTER_BOUND('',#4685,.T.);
#3352=FACE_OUTER_BOUND('',#4686,.T.);
#3353=FACE_OUTER_BOUND('',#4687,.T.);
#3354=FACE_OUTER_BOUND('',#4688,.T.);
#3355=FACE_OUTER_BOUND('',#4689,.T.);
#3356=FACE_OUTER_BOUND('',#4690,.T.);
#3357=FACE_OUTER_BOUND('',#4691,.T.);
#3358=FACE_OUTER_BOUND('',#4692,.T.);
#3359=FACE_OUTER_BOUND('',#4693,.T.);
#3360=FACE_OUTER_BOUND('',#4694,.T.);
#3361=FACE_OUTER_BOUND('',#4695,.T.);
#3362=FACE_OUTER_BOUND('',#4696,.T.);
#3363=FACE_OUTER_BOUND('',#4697,.T.);
#3364=FACE_OUTER_BOUND('',#4698,.T.);
#3365=FACE_OUTER_BOUND('',#4699,.T.);
#3366=FACE_OUTER_BOUND('',#4700,.T.);
#3367=FACE_OUTER_BOUND('',#4701,.T.);
#3368=FACE_OUTER_BOUND('',#4702,.T.);
#3369=FACE_OUTER_BOUND('',#4705,.T.);
#3370=FACE_OUTER_BOUND('',#4706,.T.);
#3371=FACE_OUTER_BOUND('',#4707,.T.);
#3372=FACE_OUTER_BOUND('',#4708,.T.);
#3373=FACE_OUTER_BOUND('',#4709,.T.);
#3374=FACE_OUTER_BOUND('',#4710,.T.);
#3375=FACE_OUTER_BOUND('',#4711,.T.);
#3376=FACE_OUTER_BOUND('',#4712,.T.);
#3377=FACE_OUTER_BOUND('',#4713,.T.);
#3378=FACE_OUTER_BOUND('',#4714,.T.);
#4332=EDGE_LOOP('',(#17835,#17836,#17837,#17838));
#4333=EDGE_LOOP('',(#17839,#17840,#17841,#17842,#17843,#17844));
#4334=EDGE_LOOP('',(#17845,#17846,#17847,#17848,#17849,#17850));
#4335=EDGE_LOOP('',(#17851,#17852,#17853,#17854,#17855,#17856));
#4336=EDGE_LOOP('',(#17857,#17858,#17859,#17860));
#4337=EDGE_LOOP('',(#17861,#17862,#17863,#17864,#17865,#17866));
#4338=EDGE_LOOP('',(#17867,#17868,#17869,#17870,#17871,#17872));
#4339=EDGE_LOOP('',(#17873,#17874,#17875,#17876,#17877,#17878));
#4340=EDGE_LOOP('',(#17879,#17880,#17881,#17882,#17883,#17884));
#4341=EDGE_LOOP('',(#17885,#17886,#17887,#17888,#17889,#17890));
#4342=EDGE_LOOP('',(#17891,#17892,#17893,#17894,#17895,#17896));
#4343=EDGE_LOOP('',(#17897,#17898,#17899,#17900,#17901,#17902));
#4344=EDGE_LOOP('',(#17903,#17904,#17905,#17906,#17907,#17908));
#4345=EDGE_LOOP('',(#17909,#17910,#17911,#17912,#17913,#17914));
#4346=EDGE_LOOP('',(#17915,#17916,#17917,#17918,#17919,#17920));
#4347=EDGE_LOOP('',(#17921,#17922,#17923,#17924,#17925,#17926));
#4348=EDGE_LOOP('',(#17927,#17928,#17929,#17930,#17931,#17932));
#4349=EDGE_LOOP('',(#17933,#17934,#17935,#17936,#17937,#17938));
#4350=EDGE_LOOP('',(#17939,#17940,#17941,#17942,#17943,#17944));
#4351=EDGE_LOOP('',(#17945,#17946,#17947,#17948,#17949,#17950));
#4352=EDGE_LOOP('',(#17951,#17952,#17953,#17954,#17955,#17956));
#4353=EDGE_LOOP('',(#17957,#17958,#17959,#17960,#17961,#17962));
#4354=EDGE_LOOP('',(#17963,#17964,#17965,#17966,#17967,#17968));
#4355=EDGE_LOOP('',(#17969,#17970,#17971,#17972,#17973,#17974));
#4356=EDGE_LOOP('',(#17975,#17976,#17977,#17978,#17979,#17980));
#4357=EDGE_LOOP('',(#17981,#17982,#17983,#17984,#17985,#17986));
#4358=EDGE_LOOP('',(#17987,#17988,#17989,#17990,#17991,#17992));
#4359=EDGE_LOOP('',(#17993,#17994,#17995,#17996,#17997,#17998));
#4360=EDGE_LOOP('',(#17999,#18000,#18001,#18002,#18003,#18004));
#4361=EDGE_LOOP('',(#18005,#18006,#18007,#18008,#18009,#18010));
#4362=EDGE_LOOP('',(#18011,#18012,#18013,#18014,#18015,#18016));
#4363=EDGE_LOOP('',(#18017,#18018,#18019,#18020,#18021,#18022));
#4364=EDGE_LOOP('',(#18023,#18024,#18025,#18026,#18027,#18028));
#4365=EDGE_LOOP('',(#18029,#18030,#18031,#18032,#18033,#18034));
#4366=EDGE_LOOP('',(#18035,#18036,#18037,#18038,#18039,#18040));
#4367=EDGE_LOOP('',(#18041,#18042,#18043,#18044,#18045,#18046));
#4368=EDGE_LOOP('',(#18047,#18048,#18049,#18050,#18051,#18052));
#4369=EDGE_LOOP('',(#18053,#18054,#18055,#18056,#18057,#18058));
#4370=EDGE_LOOP('',(#18059,#18060,#18061,#18062,#18063,#18064));
#4371=EDGE_LOOP('',(#18065,#18066,#18067,#18068,#18069,#18070));
#4372=EDGE_LOOP('',(#18071,#18072,#18073,#18074,#18075,#18076));
#4373=EDGE_LOOP('',(#18077,#18078,#18079,#18080,#18081,#18082));
#4374=EDGE_LOOP('',(#18083,#18084,#18085,#18086,#18087,#18088));
#4375=EDGE_LOOP('',(#18089,#18090,#18091,#18092,#18093,#18094));
#4376=EDGE_LOOP('',(#18095,#18096,#18097,#18098,#18099,#18100));
#4377=EDGE_LOOP('',(#18101,#18102,#18103,#18104,#18105,#18106));
#4378=EDGE_LOOP('',(#18107,#18108,#18109,#18110,#18111,#18112));
#4379=EDGE_LOOP('',(#18113,#18114,#18115,#18116,#18117,#18118));
#4380=EDGE_LOOP('',(#18119,#18120,#18121,#18122,#18123,#18124));
#4381=EDGE_LOOP('',(#18125,#18126,#18127,#18128,#18129,#18130));
#4382=EDGE_LOOP('',(#18131,#18132,#18133,#18134,#18135,#18136));
#4383=EDGE_LOOP('',(#18137,#18138,#18139,#18140,#18141,#18142));
#4384=EDGE_LOOP('',(#18143,#18144,#18145,#18146,#18147,#18148));
#4385=EDGE_LOOP('',(#18149,#18150,#18151,#18152,#18153,#18154));
#4386=EDGE_LOOP('',(#18155,#18156,#18157,#18158,#18159,#18160));
#4387=EDGE_LOOP('',(#18161,#18162,#18163,#18164,#18165,#18166));
#4388=EDGE_LOOP('',(#18167,#18168,#18169,#18170,#18171,#18172));
#4389=EDGE_LOOP('',(#18173,#18174,#18175,#18176,#18177,#18178));
#4390=EDGE_LOOP('',(#18179,#18180,#18181,#18182,#18183,#18184));
#4391=EDGE_LOOP('',(#18185,#18186,#18187,#18188,#18189,#18190));
#4392=EDGE_LOOP('',(#18191,#18192,#18193,#18194,#18195,#18196));
#4393=EDGE_LOOP('',(#18197,#18198,#18199,#18200,#18201,#18202));
#4394=EDGE_LOOP('',(#18203,#18204,#18205,#18206,#18207,#18208));
#4395=EDGE_LOOP('',(#18209,#18210,#18211,#18212,#18213,#18214));
#4396=EDGE_LOOP('',(#18215,#18216,#18217,#18218,#18219,#18220));
#4397=EDGE_LOOP('',(#18221,#18222,#18223,#18224,#18225,#18226));
#4398=EDGE_LOOP('',(#18227,#18228,#18229,#18230,#18231,#18232));
#4399=EDGE_LOOP('',(#18233,#18234,#18235,#18236,#18237,#18238));
#4400=EDGE_LOOP('',(#18239,#18240,#18241,#18242,#18243,#18244));
#4401=EDGE_LOOP('',(#18245,#18246,#18247,#18248,#18249,#18250));
#4402=EDGE_LOOP('',(#18251,#18252,#18253,#18254,#18255,#18256));
#4403=EDGE_LOOP('',(#18257,#18258,#18259,#18260,#18261,#18262));
#4404=EDGE_LOOP('',(#18263,#18264,#18265,#18266,#18267,#18268));
#4405=EDGE_LOOP('',(#18269,#18270,#18271,#18272,#18273,#18274));
#4406=EDGE_LOOP('',(#18275,#18276,#18277,#18278,#18279,#18280));
#4407=EDGE_LOOP('',(#18281,#18282,#18283,#18284,#18285,#18286));
#4408=EDGE_LOOP('',(#18287,#18288,#18289,#18290,#18291,#18292));
#4409=EDGE_LOOP('',(#18293,#18294,#18295,#18296,#18297,#18298));
#4410=EDGE_LOOP('',(#18299,#18300,#18301,#18302,#18303,#18304));
#4411=EDGE_LOOP('',(#18305,#18306,#18307,#18308,#18309,#18310));
#4412=EDGE_LOOP('',(#18311,#18312,#18313,#18314,#18315,#18316));
#4413=EDGE_LOOP('',(#18317,#18318,#18319,#18320,#18321,#18322));
#4414=EDGE_LOOP('',(#18323,#18324,#18325,#18326,#18327,#18328));
#4415=EDGE_LOOP('',(#18329,#18330,#18331,#18332,#18333,#18334));
#4416=EDGE_LOOP('',(#18335,#18336,#18337,#18338,#18339,#18340));
#4417=EDGE_LOOP('',(#18341,#18342,#18343,#18344,#18345,#18346));
#4418=EDGE_LOOP('',(#18347,#18348,#18349,#18350,#18351,#18352));
#4419=EDGE_LOOP('',(#18353,#18354,#18355,#18356,#18357,#18358));
#4420=EDGE_LOOP('',(#18359,#18360,#18361,#18362,#18363,#18364));
#4421=EDGE_LOOP('',(#18365,#18366,#18367,#18368,#18369,#18370));
#4422=EDGE_LOOP('',(#18371,#18372,#18373,#18374,#18375,#18376));
#4423=EDGE_LOOP('',(#18377,#18378,#18379,#18380,#18381,#18382));
#4424=EDGE_LOOP('',(#18383,#18384,#18385,#18386,#18387,#18388));
#4425=EDGE_LOOP('',(#18389,#18390,#18391,#18392,#18393,#18394));
#4426=EDGE_LOOP('',(#18395,#18396,#18397,#18398,#18399,#18400));
#4427=EDGE_LOOP('',(#18401,#18402,#18403,#18404,#18405,#18406));
#4428=EDGE_LOOP('',(#18407,#18408,#18409,#18410,#18411,#18412));
#4429=EDGE_LOOP('',(#18413,#18414,#18415,#18416,#18417,#18418));
#4430=EDGE_LOOP('',(#18419,#18420,#18421,#18422,#18423,#18424));
#4431=EDGE_LOOP('',(#18425,#18426,#18427,#18428,#18429,#18430));
#4432=EDGE_LOOP('',(#18431,#18432,#18433,#18434,#18435,#18436));
#4433=EDGE_LOOP('',(#18437,#18438,#18439,#18440,#18441,#18442));
#4434=EDGE_LOOP('',(#18443,#18444,#18445,#18446,#18447,#18448));
#4435=EDGE_LOOP('',(#18449,#18450,#18451,#18452,#18453,#18454));
#4436=EDGE_LOOP('',(#18455,#18456,#18457,#18458,#18459,#18460));
#4437=EDGE_LOOP('',(#18461,#18462,#18463,#18464,#18465,#18466));
#4438=EDGE_LOOP('',(#18467,#18468,#18469,#18470,#18471,#18472));
#4439=EDGE_LOOP('',(#18473,#18474,#18475,#18476,#18477,#18478));
#4440=EDGE_LOOP('',(#18479,#18480,#18481,#18482,#18483,#18484));
#4441=EDGE_LOOP('',(#18485,#18486,#18487,#18488,#18489,#18490));
#4442=EDGE_LOOP('',(#18491,#18492,#18493,#18494,#18495,#18496));
#4443=EDGE_LOOP('',(#18497,#18498,#18499,#18500,#18501,#18502));
#4444=EDGE_LOOP('',(#18503,#18504,#18505,#18506,#18507,#18508));
#4445=EDGE_LOOP('',(#18509,#18510,#18511,#18512,#18513,#18514));
#4446=EDGE_LOOP('',(#18515,#18516,#18517,#18518,#18519,#18520));
#4447=EDGE_LOOP('',(#18521,#18522,#18523,#18524,#18525,#18526));
#4448=EDGE_LOOP('',(#18527,#18528,#18529,#18530,#18531));
#4449=EDGE_LOOP('',(#18532,#18533,#18534,#18535,#18536,#18537));
#4450=EDGE_LOOP('',(#18538,#18539,#18540,#18541,#18542,#18543));
#4451=EDGE_LOOP('',(#18544,#18545,#18546));
#4452=EDGE_LOOP('',(#18547,#18548,#18549));
#4453=EDGE_LOOP('',(#18550,#18551,#18552,#18553,#18554));
#4454=EDGE_LOOP('',(#18555,#18556,#18557,#18558,#18559,#18560));
#4455=EDGE_LOOP('',(#18561,#18562,#18563,#18564,#18565));
#4456=EDGE_LOOP('',(#18566,#18567,#18568,#18569,#18570,#18571));
#4457=EDGE_LOOP('',(#18572,#18573,#18574,#18575));
#4458=EDGE_LOOP('',(#18576,#18577,#18578,#18579,#18580,#18581));
#4459=EDGE_LOOP('',(#18582,#18583,#18584,#18585,#18586));
#4460=EDGE_LOOP('',(#18587,#18588,#18589,#18590,#18591,#18592));
#4461=EDGE_LOOP('',(#18593,#18594,#18595,#18596));
#4462=EDGE_LOOP('',(#18597,#18598,#18599,#18600,#18601,#18602));
#4463=EDGE_LOOP('',(#18603,#18604,#18605,#18606));
#4464=EDGE_LOOP('',(#18607,#18608,#18609,#18610,#18611,#18612));
#4465=EDGE_LOOP('',(#18613,#18614,#18615,#18616,#18617));
#4466=EDGE_LOOP('',(#18618,#18619,#18620,#18621,#18622,#18623));
#4467=EDGE_LOOP('',(#18624,#18625,#18626,#18627,#18628));
#4468=EDGE_LOOP('',(#18629,#18630,#18631,#18632,#18633,#18634));
#4469=EDGE_LOOP('',(#18635,#18636,#18637,#18638));
#4470=EDGE_LOOP('',(#18639,#18640,#18641,#18642,#18643,#18644));
#4471=EDGE_LOOP('',(#18645,#18646,#18647,#18648,#18649));
#4472=EDGE_LOOP('',(#18650,#18651,#18652,#18653,#18654,#18655));
#4473=EDGE_LOOP('',(#18656,#18657,#18658,#18659,#18660));
#4474=EDGE_LOOP('',(#18661,#18662,#18663,#18664,#18665,#18666));
#4475=EDGE_LOOP('',(#18667,#18668,#18669,#18670));
#4476=EDGE_LOOP('',(#18671,#18672,#18673,#18674,#18675,#18676));
#4477=EDGE_LOOP('',(#18677,#18678,#18679,#18680));
#4478=EDGE_LOOP('',(#18681,#18682,#18683,#18684,#18685,#18686));
#4479=EDGE_LOOP('',(#18687,#18688,#18689,#18690,#18691));
#4480=EDGE_LOOP('',(#18692,#18693,#18694,#18695,#18696,#18697));
#4481=EDGE_LOOP('',(#18698,#18699,#18700,#18701));
#4482=EDGE_LOOP('',(#18702,#18703,#18704,#18705));
#4483=EDGE_LOOP('',(#18706,#18707,#18708,#18709,#18710,#18711));
#4484=EDGE_LOOP('',(#18712,#18713,#18714,#18715));
#4485=EDGE_LOOP('',(#18716,#18717,#18718,#18719,#18720,#18721));
#4486=EDGE_LOOP('',(#18722,#18723,#18724,#18725,#18726));
#4487=EDGE_LOOP('',(#18727,#18728,#18729,#18730,#18731,#18732));
#4488=EDGE_LOOP('',(#18733,#18734,#18735,#18736));
#4489=EDGE_LOOP('',(#18737,#18738,#18739,#18740,#18741,#18742));
#4490=EDGE_LOOP('',(#18743,#18744,#18745,#18746));
#4491=EDGE_LOOP('',(#18747,#18748,#18749,#18750,#18751,#18752));
#4492=EDGE_LOOP('',(#18753,#18754,#18755,#18756,#18757));
#4493=EDGE_LOOP('',(#18758,#18759,#18760,#18761,#18762,#18763));
#4494=EDGE_LOOP('',(#18764,#18765,#18766,#18767,#18768));
#4495=EDGE_LOOP('',(#18769,#18770,#18771,#18772,#18773,#18774));
#4496=EDGE_LOOP('',(#18775,#18776,#18777,#18778));
#4497=EDGE_LOOP('',(#18779,#18780,#18781,#18782,#18783,#18784));
#4498=EDGE_LOOP('',(#18785,#18786,#18787,#18788,#18789));
#4499=EDGE_LOOP('',(#18790,#18791,#18792,#18793,#18794,#18795));
#4500=EDGE_LOOP('',(#18796,#18797,#18798,#18799,#18800));
#4501=EDGE_LOOP('',(#18801,#18802,#18803,#18804,#18805,#18806));
#4502=EDGE_LOOP('',(#18807,#18808,#18809,#18810));
#4503=EDGE_LOOP('',(#18811,#18812,#18813,#18814,#18815,#18816));
#4504=EDGE_LOOP('',(#18817,#18818,#18819,#18820));
#4505=EDGE_LOOP('',(#18821,#18822,#18823,#18824,#18825,#18826));
#4506=EDGE_LOOP('',(#18827,#18828,#18829,#18830,#18831));
#4507=EDGE_LOOP('',(#18832,#18833,#18834,#18835,#18836,#18837));
#4508=EDGE_LOOP('',(#18838,#18839,#18840,#18841));
#4509=EDGE_LOOP('',(#18842,#18843,#18844,#18845));
#4510=EDGE_LOOP('',(#18846,#18847,#18848,#18849,#18850,#18851));
#4511=EDGE_LOOP('',(#18852,#18853,#18854,#18855));
#4512=EDGE_LOOP('',(#18856,#18857,#18858,#18859,#18860,#18861));
#4513=EDGE_LOOP('',(#18862,#18863,#18864,#18865,#18866));
#4514=EDGE_LOOP('',(#18867,#18868,#18869,#18870,#18871,#18872));
#4515=EDGE_LOOP('',(#18873,#18874,#18875,#18876));
#4516=EDGE_LOOP('',(#18877,#18878,#18879,#18880,#18881,#18882));
#4517=EDGE_LOOP('',(#18883,#18884,#18885,#18886));
#4518=EDGE_LOOP('',(#18887,#18888,#18889,#18890,#18891,#18892));
#4519=EDGE_LOOP('',(#18893,#18894,#18895,#18896,#18897));
#4520=EDGE_LOOP('',(#18898,#18899,#18900,#18901,#18902,#18903));
#4521=EDGE_LOOP('',(#18904,#18905,#18906,#18907,#18908));
#4522=EDGE_LOOP('',(#18909,#18910,#18911,#18912,#18913,#18914));
#4523=EDGE_LOOP('',(#18915,#18916,#18917,#18918));
#4524=EDGE_LOOP('',(#18919,#18920,#18921,#18922,#18923,#18924));
#4525=EDGE_LOOP('',(#18925,#18926,#18927,#18928,#18929));
#4526=EDGE_LOOP('',(#18930,#18931,#18932,#18933,#18934,#18935));
#4527=EDGE_LOOP('',(#18936,#18937,#18938,#18939,#18940));
#4528=EDGE_LOOP('',(#18941,#18942,#18943,#18944,#18945,#18946));
#4529=EDGE_LOOP('',(#18947,#18948,#18949,#18950));
#4530=EDGE_LOOP('',(#18951,#18952,#18953,#18954,#18955,#18956));
#4531=EDGE_LOOP('',(#18957,#18958,#18959,#18960));
#4532=EDGE_LOOP('',(#18961,#18962,#18963,#18964,#18965,#18966));
#4533=EDGE_LOOP('',(#18967,#18968,#18969,#18970,#18971));
#4534=EDGE_LOOP('',(#18972,#18973,#18974,#18975,#18976,#18977));
#4535=EDGE_LOOP('',(#18978,#18979,#18980,#18981));
#4536=EDGE_LOOP('',(#18982,#18983,#18984,#18985));
#4537=EDGE_LOOP('',(#18986,#18987,#18988,#18989,#18990,#18991));
#4538=EDGE_LOOP('',(#18992,#18993,#18994,#18995));
#4539=EDGE_LOOP('',(#18996,#18997,#18998,#18999,#19000,#19001));
#4540=EDGE_LOOP('',(#19002,#19003,#19004,#19005,#19006));
#4541=EDGE_LOOP('',(#19007,#19008,#19009,#19010,#19011,#19012));
#4542=EDGE_LOOP('',(#19013,#19014,#19015,#19016));
#4543=EDGE_LOOP('',(#19017,#19018,#19019,#19020,#19021,#19022));
#4544=EDGE_LOOP('',(#19023,#19024,#19025,#19026));
#4545=EDGE_LOOP('',(#19027,#19028,#19029,#19030,#19031,#19032));
#4546=EDGE_LOOP('',(#19033,#19034,#19035,#19036,#19037));
#4547=EDGE_LOOP('',(#19038,#19039,#19040,#19041,#19042,#19043));
#4548=EDGE_LOOP('',(#19044,#19045,#19046,#19047,#19048));
#4549=EDGE_LOOP('',(#19049,#19050,#19051,#19052,#19053,#19054));
#4550=EDGE_LOOP('',(#19055,#19056,#19057,#19058));
#4551=EDGE_LOOP('',(#19059,#19060,#19061,#19062,#19063,#19064));
#4552=EDGE_LOOP('',(#19065,#19066,#19067,#19068,#19069));
#4553=EDGE_LOOP('',(#19070,#19071,#19072,#19073,#19074,#19075));
#4554=EDGE_LOOP('',(#19076,#19077,#19078,#19079,#19080));
#4555=EDGE_LOOP('',(#19081,#19082,#19083,#19084,#19085,#19086));
#4556=EDGE_LOOP('',(#19087,#19088,#19089,#19090));
#4557=EDGE_LOOP('',(#19091,#19092,#19093,#19094,#19095,#19096));
#4558=EDGE_LOOP('',(#19097,#19098,#19099,#19100));
#4559=EDGE_LOOP('',(#19101,#19102,#19103,#19104,#19105,#19106));
#4560=EDGE_LOOP('',(#19107,#19108,#19109,#19110,#19111));
#4561=EDGE_LOOP('',(#19112,#19113,#19114,#19115,#19116,#19117));
#4562=EDGE_LOOP('',(#19118,#19119,#19120,#19121));
#4563=EDGE_LOOP('',(#19122,#19123,#19124,#19125));
#4564=EDGE_LOOP('',(#19126,#19127,#19128,#19129,#19130,#19131));
#4565=EDGE_LOOP('',(#19132,#19133,#19134,#19135,#19136,#19137));
#4566=EDGE_LOOP('',(#19138,#19139,#19140,#19141,#19142,#19143));
#4567=EDGE_LOOP('',(#19144,#19145,#19146,#19147,#19148,#19149));
#4568=EDGE_LOOP('',(#19150,#19151,#19152,#19153,#19154,#19155));
#4569=EDGE_LOOP('',(#19156,#19157,#19158,#19159,#19160));
#4570=EDGE_LOOP('',(#19161,#19162,#19163,#19164,#19165,#19166));
#4571=EDGE_LOOP('',(#19167,#19168,#19169,#19170,#19171,#19172));
#4572=EDGE_LOOP('',(#19173,#19174,#19175,#19176,#19177,#19178));
#4573=EDGE_LOOP('',(#19179,#19180,#19181,#19182,#19183,#19184));
#4574=EDGE_LOOP('',(#19185,#19186,#19187,#19188,#19189,#19190));
#4575=EDGE_LOOP('',(#19191,#19192,#19193,#19194,#19195,#19196));
#4576=EDGE_LOOP('',(#19197,#19198,#19199,#19200));
#4577=EDGE_LOOP('',(#19201));
#4578=EDGE_LOOP('',(#19202,#19203,#19204,#19205));
#4579=EDGE_LOOP('',(#19206,#19207,#19208,#19209,#19210));
#4580=EDGE_LOOP('',(#19211,#19212,#19213,#19214));
#4581=EDGE_LOOP('',(#19215));
#4582=EDGE_LOOP('',(#19216,#19217,#19218,#19219));
#4583=EDGE_LOOP('',(#19220,#19221,#19222,#19223,#19224));
#4584=EDGE_LOOP('',(#19225,#19226,#19227,#19228));
#4585=EDGE_LOOP('',(#19229));
#4586=EDGE_LOOP('',(#19230,#19231,#19232,#19233));
#4587=EDGE_LOOP('',(#19234,#19235,#19236,#19237,#19238,#19239));
#4588=EDGE_LOOP('',(#19240,#19241,#19242,#19243,#19244,#19245,#19246,#19247));
#4589=EDGE_LOOP('',(#19248,#19249,#19250,#19251,#19252,#19253,#19254,#19255,
#19256,#19257,#19258,#19259,#19260,#19261,#19262,#19263,#19264,#19265,#19266,
#19267,#19268,#19269,#19270,#19271,#19272,#19273,#19274,#19275,#19276,#19277,
#19278,#19279));
#4590=EDGE_LOOP('',(#19280));
#4591=EDGE_LOOP('',(#19281));
#4592=EDGE_LOOP('',(#19282,#19283,#19284,#19285));
#4593=EDGE_LOOP('',(#19286,#19287,#19288,#19289));
#4594=EDGE_LOOP('',(#19290,#19291,#19292,#19293));
#4595=EDGE_LOOP('',(#19294,#19295,#19296,#19297));
#4596=EDGE_LOOP('',(#19298));
#4597=EDGE_LOOP('',(#19299));
#4598=EDGE_LOOP('',(#19300));
#4599=EDGE_LOOP('',(#19301,#19302,#19303,#19304,#19305,#19306,#19307,#19308,
#19309,#19310,#19311,#19312,#19313,#19314,#19315,#19316,#19317,#19318));
#4600=EDGE_LOOP('',(#19319,#19320,#19321,#19322,#19323,#19324,#19325,#19326,
#19327,#19328,#19329,#19330,#19331,#19332,#19333,#19334,#19335,#19336));
#4601=EDGE_LOOP('',(#19337,#19338,#19339,#19340,#19341,#19342,#19343,#19344,
#19345,#19346,#19347,#19348,#19349,#19350,#19351,#19352,#19353,#19354));
#4602=EDGE_LOOP('',(#19355,#19356,#19357,#19358,#19359,#19360,#19361,#19362,
#19363,#19364,#19365,#19366,#19367,#19368,#19369,#19370,#19371,#19372));
#4603=EDGE_LOOP('',(#19373,#19374,#19375,#19376,#19377,#19378,#19379,#19380,
#19381,#19382,#19383,#19384,#19385,#19386,#19387,#19388,#19389,#19390,#19391,
#19392,#19393,#19394,#19395,#19396,#19397,#19398,#19399,#19400,#19401,#19402,
#19403,#19404,#19405,#19406,#19407,#19408,#19409,#19410,#19411,#19412,#19413,
#19414,#19415,#19416,#19417,#19418,#19419,#19420,#19421,#19422,#19423,#19424,
#19425,#19426,#19427,#19428,#19429,#19430,#19431,#19432,#19433,#19434,#19435,
#19436,#19437,#19438,#19439,#19440,#19441,#19442,#19443,#19444,#19445,#19446,
#19447,#19448,#19449,#19450,#19451,#19452,#19453,#19454,#19455,#19456,#19457,
#19458,#19459,#19460,#19461,#19462,#19463,#19464,#19465,#19466,#19467,#19468,
#19469,#19470,#19471,#19472,#19473,#19474,#19475));
#4604=EDGE_LOOP('',(#19476,#19477,#19478,#19479,#19480,#19481,#19482,#19483,
#19484,#19485,#19486,#19487,#19488,#19489,#19490,#19491,#19492,#19493,#19494,
#19495,#19496,#19497,#19498,#19499,#19500,#19501,#19502,#19503,#19504,#19505,
#19506,#19507,#19508,#19509,#19510,#19511,#19512,#19513,#19514,#19515,#19516,
#19517,#19518,#19519,#19520,#19521,#19522,#19523,#19524,#19525,#19526,#19527,
#19528,#19529,#19530,#19531,#19532,#19533,#19534,#19535,#19536,#19537,#19538,
#19539,#19540,#19541,#19542,#19543,#19544,#19545,#19546,#19547,#19548,#19549,
#19550,#19551,#19552,#19553,#19554,#19555,#19556,#19557,#19558,#19559,#19560,
#19561,#19562,#19563,#19564,#19565,#19566,#19567,#19568,#19569,#19570,#19571,
#19572,#19573,#19574,#19575,#19576,#19577,#19578));
#4605=EDGE_LOOP('',(#19579,#19580,#19581,#19582,#19583,#19584,#19585,#19586,
#19587,#19588,#19589,#19590,#19591,#19592,#19593,#19594,#19595,#19596,#19597,
#19598,#19599,#19600,#19601,#19602,#19603,#19604,#19605,#19606,#19607,#19608,
#19609,#19610,#19611,#19612,#19613,#19614,#19615,#19616,#19617,#19618,#19619,
#19620,#19621,#19622,#19623,#19624,#19625,#19626,#19627,#19628,#19629,#19630,
#19631,#19632,#19633,#19634,#19635,#19636,#19637,#19638,#19639,#19640,#19641,
#19642,#19643,#19644,#19645,#19646,#19647,#19648,#19649,#19650,#19651,#19652,
#19653,#19654,#19655,#19656,#19657,#19658,#19659,#19660,#19661,#19662,#19663,
#19664,#19665,#19666,#19667,#19668,#19669,#19670,#19671,#19672,#19673,#19674,
#19675,#19676,#19677,#19678,#19679,#19680,#19681));
#4606=EDGE_LOOP('',(#19682,#19683,#19684,#19685,#19686,#19687,#19688,#19689,
#19690,#19691,#19692,#19693,#19694,#19695,#19696,#19697,#19698,#19699,#19700,
#19701,#19702,#19703,#19704,#19705,#19706,#19707,#19708,#19709,#19710,#19711,
#19712,#19713,#19714,#19715,#19716,#19717,#19718,#19719,#19720,#19721,#19722,
#19723,#19724,#19725,#19726,#19727,#19728,#19729,#19730,#19731,#19732,#19733,
#19734,#19735,#19736,#19737,#19738,#19739,#19740,#19741,#19742,#19743,#19744,
#19745,#19746,#19747,#19748,#19749,#19750,#19751,#19752,#19753,#19754,#19755,
#19756,#19757,#19758,#19759,#19760,#19761,#19762,#19763,#19764,#19765,#19766,
#19767,#19768,#19769,#19770,#19771,#19772,#19773,#19774,#19775,#19776,#19777,
#19778,#19779,#19780,#19781,#19782,#19783,#19784));
#4607=EDGE_LOOP('',(#19785,#19786,#19787,#19788,#19789,#19790,#19791,#19792,
#19793,#19794,#19795,#19796,#19797,#19798,#19799,#19800,#19801,#19802,#19803,
#19804,#19805,#19806,#19807,#19808,#19809,#19810,#19811,#19812,#19813,#19814,
#19815,#19816,#19817,#19818,#19819,#19820,#19821,#19822,#19823,#19824,#19825,
#19826,#19827,#19828,#19829,#19830,#19831,#19832,#19833,#19834,#19835,#19836,
#19837,#19838,#19839,#19840,#19841,#19842,#19843,#19844,#19845,#19846,#19847,
#19848,#19849,#19850,#19851,#19852,#19853,#19854,#19855,#19856,#19857,#19858,
#19859,#19860,#19861,#19862,#19863,#19864,#19865,#19866,#19867,#19868,#19869,
#19870,#19871,#19872,#19873,#19874,#19875,#19876,#19877,#19878,#19879,#19880,
#19881,#19882,#19883,#19884,#19885,#19886,#19887));
#4608=EDGE_LOOP('',(#19888,#19889,#19890,#19891,#19892,#19893,#19894,#19895,
#19896,#19897,#19898,#19899,#19900,#19901,#19902,#19903,#19904,#19905,#19906,
#19907,#19908,#19909,#19910,#19911,#19912,#19913,#19914,#19915,#19916,#19917,
#19918,#19919,#19920,#19921,#19922,#19923,#19924,#19925,#19926,#19927,#19928,
#19929,#19930,#19931,#19932,#19933,#19934,#19935,#19936,#19937,#19938,#19939,
#19940,#19941,#19942,#19943,#19944,#19945,#19946,#19947,#19948,#19949,#19950,
#19951,#19952,#19953,#19954,#19955,#19956,#19957,#19958,#19959,#19960,#19961,
#19962,#19963,#19964,#19965,#19966,#19967,#19968,#19969,#19970,#19971,#19972,
#19973,#19974,#19975,#19976,#19977,#19978,#19979,#19980,#19981,#19982,#19983,
#19984,#19985,#19986,#19987,#19988,#19989,#19990));
#4609=EDGE_LOOP('',(#19991,#19992,#19993,#19994,#19995,#19996,#19997,#19998,
#19999,#20000,#20001,#20002,#20003,#20004,#20005,#20006,#20007,#20008,#20009,
#20010,#20011,#20012,#20013,#20014,#20015,#20016,#20017,#20018,#20019,#20020,
#20021,#20022,#20023,#20024,#20025,#20026,#20027,#20028,#20029,#20030,#20031,
#20032,#20033,#20034,#20035,#20036,#20037,#20038,#20039,#20040,#20041,#20042,
#20043,#20044,#20045,#20046,#20047,#20048,#20049,#20050,#20051,#20052,#20053,
#20054,#20055,#20056,#20057,#20058,#20059,#20060,#20061,#20062,#20063,#20064,
#20065,#20066,#20067,#20068,#20069,#20070,#20071,#20072,#20073,#20074,#20075,
#20076,#20077,#20078,#20079,#20080,#20081,#20082,#20083,#20084,#20085,#20086,
#20087,#20088,#20089,#20090,#20091,#20092,#20093));
#4610=EDGE_LOOP('',(#20094,#20095,#20096,#20097,#20098,#20099,#20100,#20101,
#20102,#20103,#20104,#20105,#20106,#20107,#20108,#20109,#20110,#20111,#20112,
#20113,#20114,#20115,#20116,#20117,#20118,#20119,#20120,#20121,#20122,#20123,
#20124,#20125,#20126,#20127,#20128,#20129,#20130,#20131,#20132,#20133,#20134,
#20135,#20136,#20137,#20138,#20139,#20140,#20141,#20142,#20143,#20144,#20145,
#20146,#20147,#20148,#20149,#20150,#20151,#20152,#20153,#20154,#20155,#20156,
#20157,#20158,#20159,#20160,#20161,#20162,#20163,#20164,#20165,#20166,#20167,
#20168,#20169,#20170,#20171,#20172,#20173,#20174,#20175,#20176,#20177,#20178,
#20179,#20180,#20181,#20182,#20183,#20184,#20185,#20186,#20187,#20188,#20189,
#20190,#20191,#20192,#20193,#20194,#20195,#20196));
#4611=EDGE_LOOP('',(#20197,#20198,#20199,#20200));
#4612=EDGE_LOOP('',(#20201,#20202,#20203,#20204));
#4613=EDGE_LOOP('',(#20205,#20206,#20207,#20208));
#4614=EDGE_LOOP('',(#20209,#20210,#20211,#20212));
#4615=EDGE_LOOP('',(#20213,#20214,#20215,#20216));
#4616=EDGE_LOOP('',(#20217,#20218,#20219,#20220));
#4617=EDGE_LOOP('',(#20221,#20222,#20223,#20224));
#4618=EDGE_LOOP('',(#20225,#20226,#20227,#20228));
#4619=EDGE_LOOP('',(#20229));
#4620=EDGE_LOOP('',(#20230,#20231,#20232,#20233,#20234,#20235,#20236));
#4621=EDGE_LOOP('',(#20237,#20238,#20239,#20240));
#4622=EDGE_LOOP('',(#20241,#20242,#20243,#20244));
#4623=EDGE_LOOP('',(#20245,#20246,#20247,#20248));
#4624=EDGE_LOOP('',(#20249,#20250,#20251,#20252));
#4625=EDGE_LOOP('',(#20253,#20254,#20255,#20256));
#4626=EDGE_LOOP('',(#20257,#20258,#20259,#20260,#20261,#20262));
#4627=EDGE_LOOP('',(#20263,#20264,#20265,#20266));
#4628=EDGE_LOOP('',(#20267));
#4629=EDGE_LOOP('',(#20268));
#4630=EDGE_LOOP('',(#20269,#20270,#20271,#20272));
#4631=EDGE_LOOP('',(#20273,#20274,#20275,#20276));
#4632=EDGE_LOOP('',(#20277,#20278,#20279,#20280));
#4633=EDGE_LOOP('',(#20281,#20282,#20283,#20284));
#4634=EDGE_LOOP('',(#20285,#20286,#20287,#20288));
#4635=EDGE_LOOP('',(#20289,#20290,#20291,#20292));
#4636=EDGE_LOOP('',(#20293,#20294,#20295,#20296));
#4637=EDGE_LOOP('',(#20297,#20298,#20299,#20300));
#4638=EDGE_LOOP('',(#20301));
#4639=EDGE_LOOP('',(#20302,#20303,#20304,#20305,#20306,#20307,#20308));
#4640=EDGE_LOOP('',(#20309,#20310,#20311,#20312,#20313,#20314,#20315));
#4641=EDGE_LOOP('',(#20316,#20317,#20318,#20319,#20320,#20321,#20322));
#4642=EDGE_LOOP('',(#20323,#20324,#20325,#20326));
#4643=EDGE_LOOP('',(#20327));
#4644=EDGE_LOOP('',(#20328,#20329,#20330,#20331,#20332));
#4645=EDGE_LOOP('',(#20333,#20334,#20335,#20336));
#4646=EDGE_LOOP('',(#20337));
#4647=EDGE_LOOP('',(#20338,#20339,#20340,#20341));
#4648=EDGE_LOOP('',(#20342,#20343,#20344,#20345));
#4649=EDGE_LOOP('',(#20346,#20347,#20348,#20349));
#4650=EDGE_LOOP('',(#20350,#20351,#20352,#20353));
#4651=EDGE_LOOP('',(#20354,#20355,#20356,#20357));
#4652=EDGE_LOOP('',(#20358,#20359,#20360,#20361,#20362,#20363));
#4653=EDGE_LOOP('',(#20364,#20365,#20366,#20367));
#4654=EDGE_LOOP('',(#20368));
#4655=EDGE_LOOP('',(#20369));
#4656=EDGE_LOOP('',(#20370,#20371,#20372,#20373));
#4657=EDGE_LOOP('',(#20374,#20375,#20376,#20377));
#4658=EDGE_LOOP('',(#20378,#20379,#20380,#20381));
#4659=EDGE_LOOP('',(#20382,#20383,#20384,#20385));
#4660=EDGE_LOOP('',(#20386,#20387,#20388,#20389));
#4661=EDGE_LOOP('',(#20390,#20391,#20392,#20393));
#4662=EDGE_LOOP('',(#20394,#20395,#20396,#20397));
#4663=EDGE_LOOP('',(#20398,#20399,#20400,#20401));
#4664=EDGE_LOOP('',(#20402));
#4665=EDGE_LOOP('',(#20403,#20404,#20405,#20406,#20407,#20408,#20409));
#4666=EDGE_LOOP('',(#20410,#20411,#20412,#20413));
#4667=EDGE_LOOP('',(#20414,#20415,#20416,#20417));
#4668=EDGE_LOOP('',(#20418,#20419,#20420,#20421));
#4669=EDGE_LOOP('',(#20422,#20423,#20424,#20425));
#4670=EDGE_LOOP('',(#20426,#20427,#20428,#20429));
#4671=EDGE_LOOP('',(#20430,#20431,#20432,#20433));
#4672=EDGE_LOOP('',(#20434,#20435,#20436,#20437));
#4673=EDGE_LOOP('',(#20438,#20439,#20440,#20441));
#4674=EDGE_LOOP('',(#20442));
#4675=EDGE_LOOP('',(#20443,#20444,#20445,#20446,#20447,#20448,#20449));
#4676=EDGE_LOOP('',(#20450,#20451,#20452,#20453,#20454,#20455,#20456));
#4677=EDGE_LOOP('',(#20457,#20458,#20459,#20460,#20461,#20462,#20463));
#4678=EDGE_LOOP('',(#20464,#20465,#20466,#20467,#20468,#20469,#20470,#20471,
#20472,#20473));
#4679=EDGE_LOOP('',(#20474));
#4680=EDGE_LOOP('',(#20475));
#4681=EDGE_LOOP('',(#20476,#20477,#20478,#20479,#20480));
#4682=EDGE_LOOP('',(#20481,#20482,#20483,#20484));
#4683=EDGE_LOOP('',(#20485));
#4684=EDGE_LOOP('',(#20486,#20487,#20488,#20489));
#4685=EDGE_LOOP('',(#20490));
#4686=EDGE_LOOP('',(#20491,#20492,#20493,#20494));
#4687=EDGE_LOOP('',(#20495));
#4688=EDGE_LOOP('',(#20496,#20497,#20498,#20499));
#4689=EDGE_LOOP('',(#20500));
#4690=EDGE_LOOP('',(#20501,#20502,#20503,#20504));
#4691=EDGE_LOOP('',(#20505,#20506,#20507,#20508));
#4692=EDGE_LOOP('',(#20509,#20510,#20511,#20512));
#4693=EDGE_LOOP('',(#20513,#20514,#20515,#20516));
#4694=EDGE_LOOP('',(#20517,#20518,#20519,#20520));
#4695=EDGE_LOOP('',(#20521,#20522,#20523,#20524));
#4696=EDGE_LOOP('',(#20525,#20526,#20527,#20528));
#4697=EDGE_LOOP('',(#20529,#20530,#20531,#20532));
#4698=EDGE_LOOP('',(#20533,#20534,#20535,#20536));
#4699=EDGE_LOOP('',(#20537,#20538,#20539,#20540));
#4700=EDGE_LOOP('',(#20541,#20542,#20543,#20544));
#4701=EDGE_LOOP('',(#20545,#20546,#20547,#20548));
#4702=EDGE_LOOP('',(#20549,#20550,#20551,#20552,#20553,#20554,#20555,#20556,
#20557,#20558));
#4703=EDGE_LOOP('',(#20559));
#4704=EDGE_LOOP('',(#20560));
#4705=EDGE_LOOP('',(#20561,#20562,#20563,#20564));
#4706=EDGE_LOOP('',(#20565,#20566,#20567,#20568));
#4707=EDGE_LOOP('',(#20569,#20570,#20571,#20572));
#4708=EDGE_LOOP('',(#20573,#20574,#20575,#20576));
#4709=EDGE_LOOP('',(#20577,#20578,#20579,#20580));
#4710=EDGE_LOOP('',(#20581,#20582,#20583,#20584));
#4711=EDGE_LOOP('',(#20585,#20586,#20587,#20588));
#4712=EDGE_LOOP('',(#20589,#20590,#20591,#20592,#20593,#20594));
#4713=EDGE_LOOP('',(#20595,#20596,#20597,#20598));
#4714=EDGE_LOOP('',(#20599,#20600,#20601,#20602,#20603,#20604,#20605,#20606,
#20607,#20608,#20609,#20610,#20611,#20612,#20613,#20614,#20615,#20616,#20617,
#20618,#20619,#20620,#20621,#20622,#20623,#20624));
#4715=EDGE_LOOP('',(#20625,#20626,#20627,#20628));
#4716=EDGE_LOOP('',(#20629,#20630,#20631,#20632));
#4717=EDGE_LOOP('',(#20633,#20634,#20635,#20636));
#4718=EDGE_LOOP('',(#20637,#20638,#20639,#20640));
#5700=CIRCLE('',#28274,5.099);
#5701=CIRCLE('',#28278,5.099);
#5702=CIRCLE('',#28280,5.099);
#5703=CIRCLE('',#28284,5.099);
#5704=CIRCLE('',#28286,2.55999999999999);
#5705=CIRCLE('',#28313,2.55999999999999);
#5706=CIRCLE('',#28315,2.56);
#5707=CIRCLE('',#28342,2.56);
#5708=CIRCLE('',#28344,2.56);
#5709=CIRCLE('',#28371,2.56);
#5710=CIRCLE('',#28373,2.56);
#5711=CIRCLE('',#28400,2.56);
#5712=CIRCLE('',#28402,4.263);
#5713=CIRCLE('',#28406,4.263);
#5714=CIRCLE('',#28408,4.263);
#5715=CIRCLE('',#28410,4.263);
#5716=CIRCLE('',#28413,4.263);
#5717=CIRCLE('',#28415,2.117);
#5718=CIRCLE('',#28442,2.117);
#5719=CIRCLE('',#28444,2.117);
#5720=CIRCLE('',#28471,2.117);
#5721=CIRCLE('',#28473,2.117);
#5722=CIRCLE('',#28500,2.117);
#5723=CIRCLE('',#28502,2.117);
#5724=CIRCLE('',#28529,2.117);
#5725=CIRCLE('',#28536,4.263);
#5726=CIRCLE('',#28544,4.);
#5727=CIRCLE('',#28545,4.);
#5728=CIRCLE('',#28548,4.5);
#5729=CIRCLE('',#28549,4.5);
#5730=CIRCLE('',#28551,3.9914370845599);
#5731=CIRCLE('',#28553,4.);
#5732=CIRCLE('',#28554,4.);
#5733=CIRCLE('',#28557,4.5);
#5734=CIRCLE('',#28558,4.5);
#5735=CIRCLE('',#28560,3.99143708455989);
#5736=CIRCLE('',#28562,5.);
#5737=CIRCLE('',#28563,5.);
#5738=CIRCLE('',#28569,0.191);
#5739=CIRCLE('',#28570,0.190999999999999);
#5740=CIRCLE('',#28571,0.253999999999999);
#5741=CIRCLE('',#28572,5.);
#5742=CIRCLE('',#28573,5.);
#5743=CIRCLE('',#28574,5.);
#5744=CIRCLE('',#28575,5.);
#5745=CIRCLE('',#28576,0.254);
#5746=CIRCLE('',#28577,0.190999999999999);
#5747=CIRCLE('',#28578,0.190999999999999);
#5748=CIRCLE('',#28579,2.5);
#5749=CIRCLE('',#28580,2.5);
#5750=CIRCLE('',#28589,3.);
#5751=CIRCLE('',#28590,3.);
#5752=CIRCLE('',#28593,6.);
#5753=CIRCLE('',#28594,6.);
#5754=CIRCLE('',#28597,6.);
#5755=CIRCLE('',#28598,6.);
#5756=CIRCLE('',#28602,4.);
#5757=CIRCLE('',#28603,5.);
#5758=CIRCLE('',#28612,3.);
#5759=CIRCLE('',#28613,3.);
#5760=CIRCLE('',#28618,4.);
#5761=CIRCLE('',#28622,5.);
#5762=CIRCLE('',#28625,6.);
#5763=CIRCLE('',#28626,6.);
#5764=CIRCLE('',#28629,6.);
#5765=CIRCLE('',#28630,6.);
#5766=CIRCLE('',#28634,4.);
#5767=CIRCLE('',#28635,5.);
#5768=CIRCLE('',#28644,3.);
#5769=CIRCLE('',#28645,3.);
#5770=CIRCLE('',#28655,3.);
#5771=CIRCLE('',#28656,3.);
#5772=CIRCLE('',#28663,5.);
#5773=CIRCLE('',#28666,4.);
#5774=CIRCLE('',#28669,2.5);
#5775=CIRCLE('',#28672,2.5);
#5776=CIRCLE('',#28676,3.99143708455989);
#5777=CIRCLE('',#28678,0.190999999999999);
#5778=CIRCLE('',#28681,0.190999999999999);
#5779=CIRCLE('',#28684,0.254);
#5780=CIRCLE('',#28687,5.);
#5781=CIRCLE('',#28689,5.);
#5782=CIRCLE('',#28692,5.);
#5783=CIRCLE('',#28695,5.);
#5784=CIRCLE('',#28698,0.253999999999999);
#5785=CIRCLE('',#28701,0.190999999999999);
#5786=CIRCLE('',#28704,0.191);
#5787=CIRCLE('',#28707,3.9914370845599);
#6413=LINE('',#36298,#8258);
#6414=LINE('',#36384,#8259);
#6415=LINE('',#36647,#8260);
#6416=LINE('',#37045,#8261);
#6417=LINE('',#37221,#8262);
#6418=LINE('',#37307,#8263);
#6419=LINE('',#37570,#8264);
#6420=LINE('',#37968,#8265);
#6421=LINE('',#38144,#8266);
#6422=LINE('',#38232,#8267);
#6423=LINE('',#38383,#8268);
#6424=LINE('',#38716,#8269);
#6425=LINE('',#38997,#8270);
#6426=LINE('',#39333,#8271);
#6427=LINE('',#39495,#8272);
#6428=LINE('',#39765,#8273);
#6429=LINE('',#40040,#8274);
#6430=LINE('',#40374,#8275);
#6431=LINE('',#40536,#8276);
#6432=LINE('',#40803,#8277);
#6433=LINE('',#41081,#8278);
#6434=LINE('',#41414,#8279);
#6435=LINE('',#41579,#8280);
#6436=LINE('',#41848,#8281);
#6437=LINE('',#42129,#8282);
#6438=LINE('',#42462,#8283);
#6439=LINE('',#42621,#8284);
#6440=LINE('',#42891,#8285);
#6441=LINE('',#43172,#8286);
#6442=LINE('',#43503,#8287);
#6443=LINE('',#43666,#8288);
#6444=LINE('',#43932,#8289);
#6445=LINE('',#44213,#8290);
#6446=LINE('',#44546,#8291);
#6447=LINE('',#44827,#8292);
#6448=LINE('',#44912,#8293);
#6449=LINE('',#45000,#8294);
#6450=LINE('',#45151,#8295);
#6451=LINE('',#45484,#8296);
#6452=LINE('',#45765,#8297);
#6453=LINE('',#46101,#8298);
#6454=LINE('',#46263,#8299);
#6455=LINE('',#46533,#8300);
#6456=LINE('',#46808,#8301);
#6457=LINE('',#47142,#8302);
#6458=LINE('',#47304,#8303);
#6459=LINE('',#47571,#8304);
#6460=LINE('',#47849,#8305);
#6461=LINE('',#48182,#8306);
#6462=LINE('',#48347,#8307);
#6463=LINE('',#48616,#8308);
#6464=LINE('',#48897,#8309);
#6465=LINE('',#49230,#8310);
#6466=LINE('',#49389,#8311);
#6467=LINE('',#49659,#8312);
#6468=LINE('',#49940,#8313);
#6469=LINE('',#50271,#8314);
#6470=LINE('',#50434,#8315);
#6471=LINE('',#50700,#8316);
#6472=LINE('',#50981,#8317);
#6473=LINE('',#51314,#8318);
#6474=LINE('',#51595,#8319);
#6475=LINE('',#51680,#8320);
#6476=LINE('',#51768,#8321);
#6477=LINE('',#51919,#8322);
#6478=LINE('',#52252,#8323);
#6479=LINE('',#52533,#8324);
#6480=LINE('',#52869,#8325);
#6481=LINE('',#53031,#8326);
#6482=LINE('',#53301,#8327);
#6483=LINE('',#53576,#8328);
#6484=LINE('',#53910,#8329);
#6485=LINE('',#54072,#8330);
#6486=LINE('',#54339,#8331);
#6487=LINE('',#54617,#8332);
#6488=LINE('',#54950,#8333);
#6489=LINE('',#55115,#8334);
#6490=LINE('',#55384,#8335);
#6491=LINE('',#55665,#8336);
#6492=LINE('',#55998,#8337);
#6493=LINE('',#56157,#8338);
#6494=LINE('',#56427,#8339);
#6495=LINE('',#56708,#8340);
#6496=LINE('',#57039,#8341);
#6497=LINE('',#57202,#8342);
#6498=LINE('',#57468,#8343);
#6499=LINE('',#57749,#8344);
#6500=LINE('',#58082,#8345);
#6501=LINE('',#58363,#8346);
#6502=LINE('',#58448,#8347);
#6503=LINE('',#58536,#8348);
#6504=LINE('',#58687,#8349);
#6505=LINE('',#59020,#8350);
#6506=LINE('',#59301,#8351);
#6507=LINE('',#59637,#8352);
#6508=LINE('',#59799,#8353);
#6509=LINE('',#60069,#8354);
#6510=LINE('',#60344,#8355);
#6511=LINE('',#60678,#8356);
#6512=LINE('',#60840,#8357);
#6513=LINE('',#61107,#8358);
#6514=LINE('',#61385,#8359);
#6515=LINE('',#61718,#8360);
#6516=LINE('',#61883,#8361);
#6517=LINE('',#62152,#8362);
#6518=LINE('',#62433,#8363);
#6519=LINE('',#62766,#8364);
#6520=LINE('',#62925,#8365);
#6521=LINE('',#63195,#8366);
#6522=LINE('',#63476,#8367);
#6523=LINE('',#63807,#8368);
#6524=LINE('',#63970,#8369);
#6525=LINE('',#64236,#8370);
#6526=LINE('',#64517,#8371);
#6527=LINE('',#64850,#8372);
#6528=LINE('',#65131,#8373);
#6529=LINE('',#65216,#8374);
#6530=LINE('',#65293,#8375);
#6531=LINE('',#65593,#8376);
#6532=LINE('',#66046,#8377);
#6533=LINE('',#66066,#8378);
#6534=LINE('',#66086,#8379);
#6535=LINE('',#66360,#8380);
#6536=LINE('',#66813,#8381);
#6537=LINE('',#66890,#8382);
#6538=LINE('',#67220,#8383);
#6539=LINE('',#67690,#8384);
#6540=LINE('',#68146,#8385);
#6541=LINE('',#68404,#8386);
#6542=LINE('',#68851,#8387);
#6543=LINE('',#69361,#8388);
#6544=LINE('',#69867,#8389);
#6545=LINE('',#70343,#8390);
#6546=LINE('',#70827,#8391);
#6547=LINE('',#71119,#8392);
#6548=LINE('',#71555,#8393);
#6549=LINE('',#71966,#8394);
#6550=LINE('',#72236,#8395);
#6551=LINE('',#72746,#8396);
#6552=LINE('',#73249,#8397);
#6553=LINE('',#73513,#8398);
#6554=LINE('',#73947,#8399);
#6555=LINE('',#74370,#8400);
#6556=LINE('',#74664,#8401);
#6557=LINE('',#75138,#8402);
#6558=LINE('',#75624,#8403);
#6559=LINE('',#76124,#8404);
#6560=LINE('',#76638,#8405);
#6561=LINE('',#77058,#8406);
#6562=LINE('',#77316,#8407);
#6563=LINE('',#77778,#8408);
#6564=LINE('',#78051,#8409);
#6565=LINE('',#78381,#8410);
#6566=LINE('',#78845,#8411);
#6567=LINE('',#79303,#8412);
#6568=LINE('',#79559,#8413);
#6569=LINE('',#80004,#8414);
#6570=LINE('',#80514,#8415);
#6571=LINE('',#81018,#8416);
#6572=LINE('',#81528,#8417);
#6573=LINE('',#82002,#8418);
#6574=LINE('',#82294,#8419);
#6575=LINE('',#82726,#8420);
#6576=LINE('',#83137,#8421);
#6577=LINE('',#83411,#8422);
#6578=LINE('',#83903,#8423);
#6579=LINE('',#84404,#8424);
#6580=LINE('',#84660,#8425);
#6581=LINE('',#85092,#8426);
#6582=LINE('',#85515,#8427);
#6583=LINE('',#85811,#8428);
#6584=LINE('',#86289,#8429);
#6585=LINE('',#86819,#8430);
#6586=LINE('',#87315,#8431);
#6587=LINE('',#87849,#8432);
#6588=LINE('',#88269,#8433);
#6589=LINE('',#88529,#8434);
#6590=LINE('',#88995,#8435);
#6591=LINE('',#89268,#8436);
#6592=LINE('',#89598,#8437);
#6593=LINE('',#90060,#8438);
#6594=LINE('',#90516,#8439);
#6595=LINE('',#90766,#8440);
#6596=LINE('',#91211,#8441);
#6597=LINE('',#91733,#8442);
#6598=LINE('',#92237,#8443);
#6599=LINE('',#92703,#8444);
#6600=LINE('',#93177,#8445);
#6601=LINE('',#93469,#8446);
#6602=LINE('',#93901,#8447);
#6603=LINE('',#94312,#8448);
#6604=LINE('',#94580,#8449);
#6605=LINE('',#95074,#8450);
#6606=LINE('',#95575,#8451);
#6607=LINE('',#95839,#8452);
#6608=LINE('',#96273,#8453);
#6609=LINE('',#96694,#8454);
#6610=LINE('',#96988,#8455);
#6611=LINE('',#97466,#8456);
#6612=LINE('',#97952,#8457);
#6613=LINE('',#98448,#8458);
#6614=LINE('',#98962,#8459);
#6615=LINE('',#99382,#8460);
#6616=LINE('',#99644,#8461);
#6617=LINE('',#100106,#8462);
#6618=LINE('',#100379,#8463);
#6619=LINE('',#100709,#8464);
#6620=LINE('',#101179,#8465);
#6621=LINE('',#101637,#8466);
#6622=LINE('',#101891,#8467);
#6623=LINE('',#102336,#8468);
#6624=LINE('',#102844,#8469);
#6625=LINE('',#103348,#8470);
#6626=LINE('',#103870,#8471);
#6627=LINE('',#104354,#8472);
#6628=LINE('',#104648,#8473);
#6629=LINE('',#105084,#8474);
#6630=LINE('',#105495,#8475);
#6631=LINE('',#105759,#8476);
#6632=LINE('',#106251,#8477);
#6633=LINE('',#106804,#8478);
#6634=LINE('',#107064,#8479);
#6635=LINE('',#107496,#8480);
#6636=LINE('',#107919,#8481);
#6637=LINE('',#108215,#8482);
#6638=LINE('',#108689,#8483);
#6639=LINE('',#109167,#8484);
#6640=LINE('',#109663,#8485);
#6641=LINE('',#110187,#8486);
#6642=LINE('',#110607,#8487);
#6643=LINE('',#110867,#8488);
#6644=LINE('',#111329,#8489);
#6645=LINE('',#115117,#8490);
#6646=LINE('',#115125,#8491);
#6647=LINE('',#115128,#8492);
#6648=LINE('',#115131,#8493);
#6649=LINE('',#115133,#8494);
#6650=LINE('',#115135,#8495);
#6651=LINE('',#115141,#8496);
#6652=LINE('',#115149,#8497);
#6653=LINE('',#115152,#8498);
#6654=LINE('',#115156,#8499);
#6655=LINE('',#115157,#8500);
#6656=LINE('',#115159,#8501);
#6657=LINE('',#115165,#8502);
#6658=LINE('',#115170,#8503);
#6659=LINE('',#115172,#8504);
#6660=LINE('',#115173,#8505);
#6661=LINE('',#115176,#8506);
#6662=LINE('',#115178,#8507);
#6663=LINE('',#115180,#8508);
#6664=LINE('',#115181,#8509);
#6665=LINE('',#115183,#8510);
#6666=LINE('',#115185,#8511);
#6667=LINE('',#115186,#8512);
#6668=LINE('',#115189,#8513);
#6669=LINE('',#115193,#8514);
#6670=LINE('',#115197,#8515);
#6671=LINE('',#115201,#8516);
#6672=LINE('',#115205,#8517);
#6673=LINE('',#115207,#8518);
#6674=LINE('',#115209,#8519);
#6675=LINE('',#115211,#8520);
#6676=LINE('',#115213,#8521);
#6677=LINE('',#115217,#8522);
#6678=LINE('',#115221,#8523);
#6679=LINE('',#115223,#8524);
#6680=LINE('',#115225,#8525);
#6681=LINE('',#115227,#8526);
#6682=LINE('',#115229,#8527);
#6683=LINE('',#115233,#8528);
#6684=LINE('',#115237,#8529);
#6685=LINE('',#115241,#8530);
#6686=LINE('',#124045,#8531);
#6687=LINE('',#124047,#8532);
#6688=LINE('',#124049,#8533);
#6689=LINE('',#124050,#8534);
#6690=LINE('',#124053,#8535);
#6691=LINE('',#124055,#8536);
#6692=LINE('',#124056,#8537);
#6693=LINE('',#124059,#8538);
#6694=LINE('',#124061,#8539);
#6695=LINE('',#124062,#8540);
#6696=LINE('',#124065,#8541);
#6697=LINE('',#124067,#8542);
#6698=LINE('',#124068,#8543);
#6699=LINE('',#124071,#8544);
#6700=LINE('',#124073,#8545);
#6701=LINE('',#124074,#8546);
#6702=LINE('',#124077,#8547);
#6703=LINE('',#124079,#8548);
#6704=LINE('',#124080,#8549);
#6705=LINE('',#124082,#8550);
#6706=LINE('',#124083,#8551);
#6707=LINE('',#124088,#8552);
#6708=LINE('',#124096,#8553);
#6709=LINE('',#124099,#8554);
#6710=LINE('',#124102,#8555);
#6711=LINE('',#124104,#8556);
#6712=LINE('',#124105,#8557);
#6713=LINE('',#124111,#8558);
#6714=LINE('',#124113,#8559);
#6715=LINE('',#124114,#8560);
#6716=LINE('',#124116,#8561);
#6717=LINE('',#124117,#8562);
#6718=LINE('',#124126,#8563);
#6719=LINE('',#124128,#8564);
#6720=LINE('',#124130,#8565);
#6721=LINE('',#124131,#8566);
#6722=LINE('',#124134,#8567);
#6723=LINE('',#124136,#8568);
#6724=LINE('',#124137,#8569);
#6725=LINE('',#124140,#8570);
#6726=LINE('',#124142,#8571);
#6727=LINE('',#124143,#8572);
#6728=LINE('',#124146,#8573);
#6729=LINE('',#124148,#8574);
#6730=LINE('',#124149,#8575);
#6731=LINE('',#124152,#8576);
#6732=LINE('',#124154,#8577);
#6733=LINE('',#124155,#8578);
#6734=LINE('',#124158,#8579);
#6735=LINE('',#124160,#8580);
#6736=LINE('',#124161,#8581);
#6737=LINE('',#124163,#8582);
#6738=LINE('',#124164,#8583);
#6739=LINE('',#124169,#8584);
#6740=LINE('',#124177,#8585);
#6741=LINE('',#124183,#8586);
#6742=LINE('',#124190,#8587);
#6743=LINE('',#124193,#8588);
#6744=LINE('',#124196,#8589);
#6745=LINE('',#124198,#8590);
#6746=LINE('',#124199,#8591);
#6747=LINE('',#124204,#8592);
#6748=LINE('',#124207,#8593);
#6749=LINE('',#124208,#8594);
#6750=LINE('',#124210,#8595);
#6751=LINE('',#124211,#8596);
#6752=LINE('',#124220,#8597);
#6753=LINE('',#124222,#8598);
#6754=LINE('',#124224,#8599);
#6755=LINE('',#124225,#8600);
#6756=LINE('',#124228,#8601);
#6757=LINE('',#124230,#8602);
#6758=LINE('',#124231,#8603);
#6759=LINE('',#124234,#8604);
#6760=LINE('',#124236,#8605);
#6761=LINE('',#124237,#8606);
#6762=LINE('',#124240,#8607);
#6763=LINE('',#124242,#8608);
#6764=LINE('',#124243,#8609);
#6765=LINE('',#124246,#8610);
#6766=LINE('',#124248,#8611);
#6767=LINE('',#124249,#8612);
#6768=LINE('',#124252,#8613);
#6769=LINE('',#124254,#8614);
#6770=LINE('',#124255,#8615);
#6771=LINE('',#124257,#8616);
#6772=LINE('',#124258,#8617);
#6773=LINE('',#124263,#8618);
#6774=LINE('',#124269,#8619);
#6775=LINE('',#124271,#8620);
#6776=LINE('',#124273,#8621);
#6777=LINE('',#124274,#8622);
#6778=LINE('',#124277,#8623);
#6779=LINE('',#124279,#8624);
#6780=LINE('',#124280,#8625);
#6781=LINE('',#124283,#8626);
#6782=LINE('',#124285,#8627);
#6783=LINE('',#124286,#8628);
#6784=LINE('',#124289,#8629);
#6785=LINE('',#124291,#8630);
#6786=LINE('',#124292,#8631);
#6787=LINE('',#124295,#8632);
#6788=LINE('',#124297,#8633);
#6789=LINE('',#124298,#8634);
#6790=LINE('',#124301,#8635);
#6791=LINE('',#124303,#8636);
#6792=LINE('',#124304,#8637);
#6793=LINE('',#124306,#8638);
#6794=LINE('',#124307,#8639);
#6795=LINE('',#124312,#8640);
#6796=LINE('',#124319,#8641);
#6797=LINE('',#124321,#8642);
#6798=LINE('',#124322,#8643);
#6799=LINE('',#124326,#8644);
#6800=LINE('',#124331,#8645);
#6801=LINE('',#124336,#8646);
#6802=LINE('',#124341,#8647);
#6803=LINE('',#124346,#8648);
#6804=LINE('',#124347,#8649);
#6805=LINE('',#124353,#8650);
#6806=LINE('',#124356,#8651);
#6807=LINE('',#124357,#8652);
#6808=LINE('',#124361,#8653);
#6809=LINE('',#124364,#8654);
#6810=LINE('',#124365,#8655);
#6811=LINE('',#124369,#8656);
#6812=LINE('',#124372,#8657);
#6813=LINE('',#124373,#8658);
#6814=LINE('',#124379,#8659);
#6815=LINE('',#124382,#8660);
#6816=LINE('',#124383,#8661);
#6817=LINE('',#124387,#8662);
#6818=LINE('',#124390,#8663);
#6819=LINE('',#124391,#8664);
#6820=LINE('',#124395,#8665);
#6821=LINE('',#124398,#8666);
#6822=LINE('',#124399,#8667);
#6823=LINE('',#124403,#8668);
#6824=LINE('',#124406,#8669);
#6825=LINE('',#124407,#8670);
#6826=LINE('',#124411,#8671);
#6827=LINE('',#124414,#8672);
#6828=LINE('',#124415,#8673);
#6829=LINE('',#124419,#8674);
#6830=LINE('',#124422,#8675);
#6831=LINE('',#124423,#8676);
#8258=VECTOR('',#30473,5.099);
#8259=VECTOR('',#30478,5.099);
#8260=VECTOR('',#30481,5.099);
#8261=VECTOR('',#30484,5.099);
#8262=VECTOR('',#30489,5.099);
#8263=VECTOR('',#30494,5.099);
#8264=VECTOR('',#30497,5.099);
#8265=VECTOR('',#30500,5.099);
#8266=VECTOR('',#30505,2.55999999999999);
#8267=VECTOR('',#30510,2.55999999999999);
#8268=VECTOR('',#30513,2.55999999999999);
#8269=VECTOR('',#30516,2.55999999999999);
#8270=VECTOR('',#30519,2.55999999999999);
#8271=VECTOR('',#30522,2.55999999999999);
#8272=VECTOR('',#30525,2.55999999999999);
#8273=VECTOR('',#30528,2.55999999999999);
#8274=VECTOR('',#30531,2.55999999999999);
#8275=VECTOR('',#30534,2.55999999999999);
#8276=VECTOR('',#30537,2.55999999999999);
#8277=VECTOR('',#30540,2.55999999999999);
#8278=VECTOR('',#30543,2.55999999999999);
#8279=VECTOR('',#30546,2.55999999999999);
#8280=VECTOR('',#30549,2.55999999999999);
#8281=VECTOR('',#30552,2.55999999999999);
#8282=VECTOR('',#30555,2.55999999999999);
#8283=VECTOR('',#30558,2.55999999999999);
#8284=VECTOR('',#30561,2.55999999999999);
#8285=VECTOR('',#30564,2.55999999999999);
#8286=VECTOR('',#30567,2.55999999999999);
#8287=VECTOR('',#30570,2.55999999999999);
#8288=VECTOR('',#30573,2.55999999999999);
#8289=VECTOR('',#30576,2.55999999999999);
#8290=VECTOR('',#30579,2.55999999999999);
#8291=VECTOR('',#30582,2.55999999999999);
#8292=VECTOR('',#30585,2.55999999999999);
#8293=VECTOR('',#30590,2.56);
#8294=VECTOR('',#30595,2.56);
#8295=VECTOR('',#30598,2.56);
#8296=VECTOR('',#30601,2.56);
#8297=VECTOR('',#30604,2.56);
#8298=VECTOR('',#30607,2.56);
#8299=VECTOR('',#30610,2.56);
#8300=VECTOR('',#30613,2.56);
#8301=VECTOR('',#30616,2.56);
#8302=VECTOR('',#30619,2.56);
#8303=VECTOR('',#30622,2.56);
#8304=VECTOR('',#30625,2.56);
#8305=VECTOR('',#30628,2.56);
#8306=VECTOR('',#30631,2.56);
#8307=VECTOR('',#30634,2.56);
#8308=VECTOR('',#30637,2.56);
#8309=VECTOR('',#30640,2.56);
#8310=VECTOR('',#30643,2.56);
#8311=VECTOR('',#30646,2.56);
#8312=VECTOR('',#30649,2.56);
#8313=VECTOR('',#30652,2.56);
#8314=VECTOR('',#30655,2.56);
#8315=VECTOR('',#30658,2.56);
#8316=VECTOR('',#30661,2.56);
#8317=VECTOR('',#30664,2.56);
#8318=VECTOR('',#30667,2.56);
#8319=VECTOR('',#30670,2.56);
#8320=VECTOR('',#30675,2.56);
#8321=VECTOR('',#30680,2.56);
#8322=VECTOR('',#30683,2.56);
#8323=VECTOR('',#30686,2.56);
#8324=VECTOR('',#30689,2.56);
#8325=VECTOR('',#30692,2.56);
#8326=VECTOR('',#30695,2.56);
#8327=VECTOR('',#30698,2.56);
#8328=VECTOR('',#30701,2.56);
#8329=VECTOR('',#30704,2.56);
#8330=VECTOR('',#30707,2.56);
#8331=VECTOR('',#30710,2.56);
#8332=VECTOR('',#30713,2.56);
#8333=VECTOR('',#30716,2.56);
#8334=VECTOR('',#30719,2.56);
#8335=VECTOR('',#30722,2.56);
#8336=VECTOR('',#30725,2.56);
#8337=VECTOR('',#30728,2.56);
#8338=VECTOR('',#30731,2.56);
#8339=VECTOR('',#30734,2.56);
#8340=VECTOR('',#30737,2.56);
#8341=VECTOR('',#30740,2.56);
#8342=VECTOR('',#30743,2.56);
#8343=VECTOR('',#30746,2.56);
#8344=VECTOR('',#30749,2.56);
#8345=VECTOR('',#30752,2.56);
#8346=VECTOR('',#30755,2.56);
#8347=VECTOR('',#30760,2.56);
#8348=VECTOR('',#30765,2.56);
#8349=VECTOR('',#30768,2.56);
#8350=VECTOR('',#30771,2.56);
#8351=VECTOR('',#30774,2.56);
#8352=VECTOR('',#30777,2.56);
#8353=VECTOR('',#30780,2.56);
#8354=VECTOR('',#30783,2.56);
#8355=VECTOR('',#30786,2.56);
#8356=VECTOR('',#30789,2.56);
#8357=VECTOR('',#30792,2.56);
#8358=VECTOR('',#30795,2.56);
#8359=VECTOR('',#30798,2.56);
#8360=VECTOR('',#30801,2.56);
#8361=VECTOR('',#30804,2.56);
#8362=VECTOR('',#30807,2.56);
#8363=VECTOR('',#30810,2.56);
#8364=VECTOR('',#30813,2.56);
#8365=VECTOR('',#30816,2.56);
#8366=VECTOR('',#30819,2.56);
#8367=VECTOR('',#30822,2.56);
#8368=VECTOR('',#30825,2.56);
#8369=VECTOR('',#30828,2.56);
#8370=VECTOR('',#30831,2.56);
#8371=VECTOR('',#30834,2.56);
#8372=VECTOR('',#30837,2.56);
#8373=VECTOR('',#30840,2.56);
#8374=VECTOR('',#30845,4.263);
#8375=VECTOR('',#30850,4.263);
#8376=VECTOR('',#30853,4.263);
#8377=VECTOR('',#30856,4.263);
#8378=VECTOR('',#30861,4.263);
#8379=VECTOR('',#30866,4.263);
#8380=VECTOR('',#30871,4.263);
#8381=VECTOR('',#30874,4.263);
#8382=VECTOR('',#30879,2.117);
#8383=VECTOR('',#30884,2.117);
#8384=VECTOR('',#30887,2.117);
#8385=VECTOR('',#30890,2.117);
#8386=VECTOR('',#30893,2.117);
#8387=VECTOR('',#30896,2.117);
#8388=VECTOR('',#30899,2.117);
#8389=VECTOR('',#30902,2.117);
#8390=VECTOR('',#30905,2.117);
#8391=VECTOR('',#30908,2.117);
#8392=VECTOR('',#30911,2.117);
#8393=VECTOR('',#30914,2.117);
#8394=VECTOR('',#30917,2.117);
#8395=VECTOR('',#30920,2.117);
#8396=VECTOR('',#30923,2.117);
#8397=VECTOR('',#30926,2.117);
#8398=VECTOR('',#30929,2.117);
#8399=VECTOR('',#30932,2.117);
#8400=VECTOR('',#30935,2.117);
#8401=VECTOR('',#30938,2.117);
#8402=VECTOR('',#30941,2.117);
#8403=VECTOR('',#30944,2.117);
#8404=VECTOR('',#30947,2.117);
#8405=VECTOR('',#30950,2.117);
#8406=VECTOR('',#30953,2.117);
#8407=VECTOR('',#30956,2.117);
#8408=VECTOR('',#30959,2.117);
#8409=VECTOR('',#30964,2.117);
#8410=VECTOR('',#30969,2.117);
#8411=VECTOR('',#30972,2.117);
#8412=VECTOR('',#30975,2.117);
#8413=VECTOR('',#30978,2.117);
#8414=VECTOR('',#30981,2.117);
#8415=VECTOR('',#30984,2.117);
#8416=VECTOR('',#30987,2.117);
#8417=VECTOR('',#30990,2.117);
#8418=VECTOR('',#30993,2.117);
#8419=VECTOR('',#30996,2.117);
#8420=VECTOR('',#30999,2.117);
#8421=VECTOR('',#31002,2.117);
#8422=VECTOR('',#31005,2.117);
#8423=VECTOR('',#31008,2.117);
#8424=VECTOR('',#31011,2.117);
#8425=VECTOR('',#31014,2.117);
#8426=VECTOR('',#31017,2.117);
#8427=VECTOR('',#31020,2.117);
#8428=VECTOR('',#31023,2.117);
#8429=VECTOR('',#31026,2.117);
#8430=VECTOR('',#31029,2.117);
#8431=VECTOR('',#31032,2.117);
#8432=VECTOR('',#31035,2.117);
#8433=VECTOR('',#31038,2.117);
#8434=VECTOR('',#31041,2.117);
#8435=VECTOR('',#31044,2.117);
#8436=VECTOR('',#31049,2.117);
#8437=VECTOR('',#31054,2.117);
#8438=VECTOR('',#31057,2.117);
#8439=VECTOR('',#31060,2.117);
#8440=VECTOR('',#31063,2.117);
#8441=VECTOR('',#31066,2.117);
#8442=VECTOR('',#31069,2.117);
#8443=VECTOR('',#31072,2.117);
#8444=VECTOR('',#31075,2.117);
#8445=VECTOR('',#31078,2.117);
#8446=VECTOR('',#31081,2.117);
#8447=VECTOR('',#31084,2.117);
#8448=VECTOR('',#31087,2.117);
#8449=VECTOR('',#31090,2.117);
#8450=VECTOR('',#31093,2.117);
#8451=VECTOR('',#31096,2.117);
#8452=VECTOR('',#31099,2.117);
#8453=VECTOR('',#31102,2.117);
#8454=VECTOR('',#31105,2.117);
#8455=VECTOR('',#31108,2.117);
#8456=VECTOR('',#31111,2.117);
#8457=VECTOR('',#31114,2.117);
#8458=VECTOR('',#31117,2.117);
#8459=VECTOR('',#31120,2.117);
#8460=VECTOR('',#31123,2.117);
#8461=VECTOR('',#31126,2.117);
#8462=VECTOR('',#31129,2.117);
#8463=VECTOR('',#31134,2.117);
#8464=VECTOR('',#31139,2.117);
#8465=VECTOR('',#31142,2.117);
#8466=VECTOR('',#31145,2.117);
#8467=VECTOR('',#31148,2.117);
#8468=VECTOR('',#31151,2.117);
#8469=VECTOR('',#31154,2.117);
#8470=VECTOR('',#31157,2.117);
#8471=VECTOR('',#31160,2.117);
#8472=VECTOR('',#31163,2.117);
#8473=VECTOR('',#31166,2.117);
#8474=VECTOR('',#31169,2.117);
#8475=VECTOR('',#31172,2.117);
#8476=VECTOR('',#31175,2.117);
#8477=VECTOR('',#31178,2.117);
#8478=VECTOR('',#31181,2.117);
#8479=VECTOR('',#31184,2.117);
#8480=VECTOR('',#31187,2.117);
#8481=VECTOR('',#31190,2.117);
#8482=VECTOR('',#31193,2.117);
#8483=VECTOR('',#31196,2.117);
#8484=VECTOR('',#31199,2.117);
#8485=VECTOR('',#31202,2.117);
#8486=VECTOR('',#31205,2.117);
#8487=VECTOR('',#31208,2.117);
#8488=VECTOR('',#31211,2.117);
#8489=VECTOR('',#31214,2.117);
#8490=VECTOR('',#31247,4.);
#8491=VECTOR('',#31256,10.);
#8492=VECTOR('',#31259,10.);
#8493=VECTOR('',#31262,10.);
#8494=VECTOR('',#31263,10.);
#8495=VECTOR('',#31264,10.);
#8496=VECTOR('',#31271,4.);
#8497=VECTOR('',#31280,10.);
#8498=VECTOR('',#31283,10.);
#8499=VECTOR('',#31286,10.);
#8500=VECTOR('',#31287,10.);
#8501=VECTOR('',#31288,10.);
#8502=VECTOR('',#31295,5.);
#8503=VECTOR('',#31302,10.);
#8504=VECTOR('',#31303,10.);
#8505=VECTOR('',#31304,10.);
#8506=VECTOR('',#31307,10.);
#8507=VECTOR('',#31308,10.);
#8508=VECTOR('',#31309,10.);
#8509=VECTOR('',#31310,10.);
#8510=VECTOR('',#31313,10.);
#8511=VECTOR('',#31314,10.);
#8512=VECTOR('',#31315,10.);
#8513=VECTOR('',#31318,10.);
#8514=VECTOR('',#31321,10.);
#8515=VECTOR('',#31324,10.);
#8516=VECTOR('',#31327,10.);
#8517=VECTOR('',#31330,10.);
#8518=VECTOR('',#31331,10.);
#8519=VECTOR('',#31332,10.);
#8520=VECTOR('',#31333,10.);
#8521=VECTOR('',#31334,10.);
#8522=VECTOR('',#31337,10.);
#8523=VECTOR('',#31340,10.);
#8524=VECTOR('',#31341,10.);
#8525=VECTOR('',#31342,10.);
#8526=VECTOR('',#31343,10.);
#8527=VECTOR('',#31344,10.);
#8528=VECTOR('',#31347,10.);
#8529=VECTOR('',#31350,10.);
#8530=VECTOR('',#31353,10.);
#8531=VECTOR('',#31362,10.);
#8532=VECTOR('',#31363,10.);
#8533=VECTOR('',#31364,10.);
#8534=VECTOR('',#31365,10.);
#8535=VECTOR('',#31368,10.);
#8536=VECTOR('',#31369,10.);
#8537=VECTOR('',#31370,10.);
#8538=VECTOR('',#31373,10.);
#8539=VECTOR('',#31374,10.);
#8540=VECTOR('',#31375,10.);
#8541=VECTOR('',#31378,10.);
#8542=VECTOR('',#31379,10.);
#8543=VECTOR('',#31380,10.);
#8544=VECTOR('',#31383,10.);
#8545=VECTOR('',#31384,10.);
#8546=VECTOR('',#31385,10.);
#8547=VECTOR('',#31388,10.);
#8548=VECTOR('',#31389,10.);
#8549=VECTOR('',#31390,10.);
#8550=VECTOR('',#31393,10.);
#8551=VECTOR('',#31394,10.);
#8552=VECTOR('',#31399,3.);
#8553=VECTOR('',#31408,10.);
#8554=VECTOR('',#31411,10.);
#8555=VECTOR('',#31414,10.);
#8556=VECTOR('',#31415,10.);
#8557=VECTOR('',#31416,10.);
#8558=VECTOR('',#31423,10.);
#8559=VECTOR('',#31426,10.);
#8560=VECTOR('',#31427,10.);
#8561=VECTOR('',#31430,10.);
#8562=VECTOR('',#31431,10.);
#8563=VECTOR('',#31440,10.);
#8564=VECTOR('',#31441,10.);
#8565=VECTOR('',#31442,10.);
#8566=VECTOR('',#31443,10.);
#8567=VECTOR('',#31446,10.);
#8568=VECTOR('',#31447,10.);
#8569=VECTOR('',#31448,10.);
#8570=VECTOR('',#31451,10.);
#8571=VECTOR('',#31452,10.);
#8572=VECTOR('',#31453,10.);
#8573=VECTOR('',#31456,10.);
#8574=VECTOR('',#31457,10.);
#8575=VECTOR('',#31458,10.);
#8576=VECTOR('',#31461,10.);
#8577=VECTOR('',#31462,10.);
#8578=VECTOR('',#31463,10.);
#8579=VECTOR('',#31466,10.);
#8580=VECTOR('',#31467,10.);
#8581=VECTOR('',#31468,10.);
#8582=VECTOR('',#31471,10.);
#8583=VECTOR('',#31472,10.);
#8584=VECTOR('',#31477,3.);
#8585=VECTOR('',#31490,4.);
#8586=VECTOR('',#31499,5.);
#8587=VECTOR('',#31506,10.);
#8588=VECTOR('',#31509,10.);
#8589=VECTOR('',#31512,10.);
#8590=VECTOR('',#31513,10.);
#8591=VECTOR('',#31514,10.);
#8592=VECTOR('',#31519,10.);
#8593=VECTOR('',#31524,10.);
#8594=VECTOR('',#31525,10.);
#8595=VECTOR('',#31528,10.);
#8596=VECTOR('',#31529,10.);
#8597=VECTOR('',#31538,10.);
#8598=VECTOR('',#31539,10.);
#8599=VECTOR('',#31540,10.);
#8600=VECTOR('',#31541,10.);
#8601=VECTOR('',#31544,10.);
#8602=VECTOR('',#31545,10.);
#8603=VECTOR('',#31546,10.);
#8604=VECTOR('',#31549,10.);
#8605=VECTOR('',#31550,10.);
#8606=VECTOR('',#31551,10.);
#8607=VECTOR('',#31554,10.);
#8608=VECTOR('',#31555,10.);
#8609=VECTOR('',#31556,10.);
#8610=VECTOR('',#31559,10.);
#8611=VECTOR('',#31560,10.);
#8612=VECTOR('',#31561,10.);
#8613=VECTOR('',#31564,10.);
#8614=VECTOR('',#31565,10.);
#8615=VECTOR('',#31566,10.);
#8616=VECTOR('',#31569,10.);
#8617=VECTOR('',#31570,10.);
#8618=VECTOR('',#31575,3.);
#8619=VECTOR('',#31582,10.);
#8620=VECTOR('',#31583,10.);
#8621=VECTOR('',#31584,10.);
#8622=VECTOR('',#31585,10.);
#8623=VECTOR('',#31588,10.);
#8624=VECTOR('',#31589,10.);
#8625=VECTOR('',#31590,10.);
#8626=VECTOR('',#31593,10.);
#8627=VECTOR('',#31594,10.);
#8628=VECTOR('',#31595,10.);
#8629=VECTOR('',#31598,10.);
#8630=VECTOR('',#31599,10.);
#8631=VECTOR('',#31600,10.);
#8632=VECTOR('',#31603,10.);
#8633=VECTOR('',#31604,10.);
#8634=VECTOR('',#31605,10.);
#8635=VECTOR('',#31608,10.);
#8636=VECTOR('',#31609,10.);
#8637=VECTOR('',#31610,10.);
#8638=VECTOR('',#31613,10.);
#8639=VECTOR('',#31614,10.);
#8640=VECTOR('',#31619,3.);
#8641=VECTOR('',#31630,10.);
#8642=VECTOR('',#31631,10.);
#8643=VECTOR('',#31632,10.);
#8644=VECTOR('',#31637,5.);
#8645=VECTOR('',#31644,4.);
#8646=VECTOR('',#31651,2.5);
#8647=VECTOR('',#31658,2.5);
#8648=VECTOR('',#31665,10.);
#8649=VECTOR('',#31666,10.);
#8650=VECTOR('',#31675,10.);
#8651=VECTOR('',#31678,10.);
#8652=VECTOR('',#31679,10.);
#8653=VECTOR('',#31684,10.);
#8654=VECTOR('',#31687,10.);
#8655=VECTOR('',#31688,10.);
#8656=VECTOR('',#31693,10.);
#8657=VECTOR('',#31696,10.);
#8658=VECTOR('',#31697,10.);
#8659=VECTOR('',#31706,10.);
#8660=VECTOR('',#31709,10.);
#8661=VECTOR('',#31710,10.);
#8662=VECTOR('',#31715,10.);
#8663=VECTOR('',#31718,10.);
#8664=VECTOR('',#31719,10.);
#8665=VECTOR('',#31724,10.);
#8666=VECTOR('',#31727,10.);
#8667=VECTOR('',#31728,10.);
#8668=VECTOR('',#31733,10.);
#8669=VECTOR('',#31736,10.);
#8670=VECTOR('',#31737,10.);
#8671=VECTOR('',#31742,10.);
#8672=VECTOR('',#31745,10.);
#8673=VECTOR('',#31746,10.);
#8674=VECTOR('',#31751,10.);
#8675=VECTOR('',#31754,10.);
#8676=VECTOR('',#31755,10.);
#10088=VERTEX_POINT('',#36296);
#10089=VERTEX_POINT('',#36297);
#10090=VERTEX_POINT('',#36299);
#10091=VERTEX_POINT('',#36306);
#10092=VERTEX_POINT('',#36382);
#10093=VERTEX_POINT('',#36383);
#10094=VERTEX_POINT('',#36385);
#10095=VERTEX_POINT('',#36546);
#10096=VERTEX_POINT('',#36645);
#10097=VERTEX_POINT('',#36646);
#10098=VERTEX_POINT('',#36648);
#10099=VERTEX_POINT('',#36885);
#10100=VERTEX_POINT('',#37043);
#10101=VERTEX_POINT('',#37044);
#10102=VERTEX_POINT('',#37046);
#10103=VERTEX_POINT('',#37132);
#10104=VERTEX_POINT('',#37139);
#10105=VERTEX_POINT('',#37141);
#10106=VERTEX_POINT('',#37219);
#10107=VERTEX_POINT('',#37220);
#10108=VERTEX_POINT('',#37222);
#10109=VERTEX_POINT('',#37229);
#10110=VERTEX_POINT('',#37305);
#10111=VERTEX_POINT('',#37306);
#10112=VERTEX_POINT('',#37308);
#10113=VERTEX_POINT('',#37469);
#10114=VERTEX_POINT('',#37568);
#10115=VERTEX_POINT('',#37569);
#10116=VERTEX_POINT('',#37571);
#10117=VERTEX_POINT('',#37808);
#10118=VERTEX_POINT('',#37966);
#10119=VERTEX_POINT('',#37967);
#10120=VERTEX_POINT('',#37969);
#10121=VERTEX_POINT('',#38055);
#10122=VERTEX_POINT('',#38062);
#10123=VERTEX_POINT('',#38064);
#10124=VERTEX_POINT('',#38142);
#10125=VERTEX_POINT('',#38143);
#10126=VERTEX_POINT('',#38145);
#10127=VERTEX_POINT('',#38154);
#10128=VERTEX_POINT('',#38160);
#10129=VERTEX_POINT('',#38162);
#10130=VERTEX_POINT('',#38230);
#10131=VERTEX_POINT('',#38231);
#10132=VERTEX_POINT('',#38233);
#10133=VERTEX_POINT('',#38364);
#10134=VERTEX_POINT('',#38381);
#10135=VERTEX_POINT('',#38382);
#10136=VERTEX_POINT('',#38384);
#10137=VERTEX_POINT('',#38582);
#10138=VERTEX_POINT('',#38714);
#10139=VERTEX_POINT('',#38715);
#10140=VERTEX_POINT('',#38717);
#10141=VERTEX_POINT('',#38796);
#10142=VERTEX_POINT('',#38995);
#10143=VERTEX_POINT('',#38996);
#10144=VERTEX_POINT('',#38998);
#10145=VERTEX_POINT('',#39132);
#10146=VERTEX_POINT('',#39331);
#10147=VERTEX_POINT('',#39332);
#10148=VERTEX_POINT('',#39334);
#10149=VERTEX_POINT('',#39413);
#10150=VERTEX_POINT('',#39493);
#10151=VERTEX_POINT('',#39494);
#10152=VERTEX_POINT('',#39496);
#10153=VERTEX_POINT('',#39631);
#10154=VERTEX_POINT('',#39763);
#10155=VERTEX_POINT('',#39764);
#10156=VERTEX_POINT('',#39766);
#10157=VERTEX_POINT('',#39958);
#10158=VERTEX_POINT('',#40038);
#10159=VERTEX_POINT('',#40039);
#10160=VERTEX_POINT('',#40041);
#10161=VERTEX_POINT('',#40236);
#10162=VERTEX_POINT('',#40372);
#10163=VERTEX_POINT('',#40373);
#10164=VERTEX_POINT('',#40375);
#10165=VERTEX_POINT('',#40454);
#10166=VERTEX_POINT('',#40534);
#10167=VERTEX_POINT('',#40535);
#10168=VERTEX_POINT('',#40537);
#10169=VERTEX_POINT('',#40669);
#10170=VERTEX_POINT('',#40801);
#10171=VERTEX_POINT('',#40802);
#10172=VERTEX_POINT('',#40804);
#10173=VERTEX_POINT('',#40999);
#10174=VERTEX_POINT('',#41079);
#10175=VERTEX_POINT('',#41080);
#10176=VERTEX_POINT('',#41082);
#10177=VERTEX_POINT('',#41280);
#10178=VERTEX_POINT('',#41412);
#10179=VERTEX_POINT('',#41413);
#10180=VERTEX_POINT('',#41415);
#10181=VERTEX_POINT('',#41494);
#10182=VERTEX_POINT('',#41577);
#10183=VERTEX_POINT('',#41578);
#10184=VERTEX_POINT('',#41580);
#10185=VERTEX_POINT('',#41714);
#10186=VERTEX_POINT('',#41846);
#10187=VERTEX_POINT('',#41847);
#10188=VERTEX_POINT('',#41849);
#10189=VERTEX_POINT('',#41928);
#10190=VERTEX_POINT('',#42127);
#10191=VERTEX_POINT('',#42128);
#10192=VERTEX_POINT('',#42130);
#10193=VERTEX_POINT('',#42264);
#10194=VERTEX_POINT('',#42460);
#10195=VERTEX_POINT('',#42461);
#10196=VERTEX_POINT('',#42463);
#10197=VERTEX_POINT('',#42539);
#10198=VERTEX_POINT('',#42619);
#10199=VERTEX_POINT('',#42620);
#10200=VERTEX_POINT('',#42622);
#10201=VERTEX_POINT('',#42753);
#10202=VERTEX_POINT('',#42889);
#10203=VERTEX_POINT('',#42890);
#10204=VERTEX_POINT('',#42892);
#10205=VERTEX_POINT('',#42971);
#10206=VERTEX_POINT('',#43170);
#10207=VERTEX_POINT('',#43171);
#10208=VERTEX_POINT('',#43173);
#10209=VERTEX_POINT('',#43305);
#10210=VERTEX_POINT('',#43501);
#10211=VERTEX_POINT('',#43502);
#10212=VERTEX_POINT('',#43504);
#10213=VERTEX_POINT('',#43583);
#10214=VERTEX_POINT('',#43664);
#10215=VERTEX_POINT('',#43665);
#10216=VERTEX_POINT('',#43667);
#10217=VERTEX_POINT('',#43798);
#10218=VERTEX_POINT('',#43930);
#10219=VERTEX_POINT('',#43931);
#10220=VERTEX_POINT('',#43933);
#10221=VERTEX_POINT('',#44131);
#10222=VERTEX_POINT('',#44211);
#10223=VERTEX_POINT('',#44212);
#10224=VERTEX_POINT('',#44214);
#10225=VERTEX_POINT('',#44412);
#10226=VERTEX_POINT('',#44544);
#10227=VERTEX_POINT('',#44545);
#10228=VERTEX_POINT('',#44547);
#10229=VERTEX_POINT('',#44626);
#10230=VERTEX_POINT('',#44825);
#10231=VERTEX_POINT('',#44826);
#10232=VERTEX_POINT('',#44828);
#10233=VERTEX_POINT('',#44835);
#10234=VERTEX_POINT('',#44841);
#10235=VERTEX_POINT('',#44843);
#10236=VERTEX_POINT('',#44910);
#10237=VERTEX_POINT('',#44911);
#10238=VERTEX_POINT('',#44913);
#10239=VERTEX_POINT('',#44922);
#10240=VERTEX_POINT('',#44928);
#10241=VERTEX_POINT('',#44930);
#10242=VERTEX_POINT('',#44998);
#10243=VERTEX_POINT('',#44999);
#10244=VERTEX_POINT('',#45001);
#10245=VERTEX_POINT('',#45132);
#10246=VERTEX_POINT('',#45149);
#10247=VERTEX_POINT('',#45150);
#10248=VERTEX_POINT('',#45152);
#10249=VERTEX_POINT('',#45350);
#10250=VERTEX_POINT('',#45482);
#10251=VERTEX_POINT('',#45483);
#10252=VERTEX_POINT('',#45485);
#10253=VERTEX_POINT('',#45564);
#10254=VERTEX_POINT('',#45763);
#10255=VERTEX_POINT('',#45764);
#10256=VERTEX_POINT('',#45766);
#10257=VERTEX_POINT('',#45900);
#10258=VERTEX_POINT('',#46099);
#10259=VERTEX_POINT('',#46100);
#10260=VERTEX_POINT('',#46102);
#10261=VERTEX_POINT('',#46181);
#10262=VERTEX_POINT('',#46261);
#10263=VERTEX_POINT('',#46262);
#10264=VERTEX_POINT('',#46264);
#10265=VERTEX_POINT('',#46399);
#10266=VERTEX_POINT('',#46531);
#10267=VERTEX_POINT('',#46532);
#10268=VERTEX_POINT('',#46534);
#10269=VERTEX_POINT('',#46726);
#10270=VERTEX_POINT('',#46806);
#10271=VERTEX_POINT('',#46807);
#10272=VERTEX_POINT('',#46809);
#10273=VERTEX_POINT('',#47004);
#10274=VERTEX_POINT('',#47140);
#10275=VERTEX_POINT('',#47141);
#10276=VERTEX_POINT('',#47143);
#10277=VERTEX_POINT('',#47222);
#10278=VERTEX_POINT('',#47302);
#10279=VERTEX_POINT('',#47303);
#10280=VERTEX_POINT('',#47305);
#10281=VERTEX_POINT('',#47437);
#10282=VERTEX_POINT('',#47569);
#10283=VERTEX_POINT('',#47570);
#10284=VERTEX_POINT('',#47572);
#10285=VERTEX_POINT('',#47767);
#10286=VERTEX_POINT('',#47847);
#10287=VERTEX_POINT('',#47848);
#10288=VERTEX_POINT('',#47850);
#10289=VERTEX_POINT('',#48048);
#10290=VERTEX_POINT('',#48180);
#10291=VERTEX_POINT('',#48181);
#10292=VERTEX_POINT('',#48183);
#10293=VERTEX_POINT('',#48262);
#10294=VERTEX_POINT('',#48345);
#10295=VERTEX_POINT('',#48346);
#10296=VERTEX_POINT('',#48348);
#10297=VERTEX_POINT('',#48482);
#10298=VERTEX_POINT('',#48614);
#10299=VERTEX_POINT('',#48615);
#10300=VERTEX_POINT('',#48617);
#10301=VERTEX_POINT('',#48696);
#10302=VERTEX_POINT('',#48895);
#10303=VERTEX_POINT('',#48896);
#10304=VERTEX_POINT('',#48898);
#10305=VERTEX_POINT('',#49032);
#10306=VERTEX_POINT('',#49228);
#10307=VERTEX_POINT('',#49229);
#10308=VERTEX_POINT('',#49231);
#10309=VERTEX_POINT('',#49307);
#10310=VERTEX_POINT('',#49387);
#10311=VERTEX_POINT('',#49388);
#10312=VERTEX_POINT('',#49390);
#10313=VERTEX_POINT('',#49521);
#10314=VERTEX_POINT('',#49657);
#10315=VERTEX_POINT('',#49658);
#10316=VERTEX_POINT('',#49660);
#10317=VERTEX_POINT('',#49739);
#10318=VERTEX_POINT('',#49938);
#10319=VERTEX_POINT('',#49939);
#10320=VERTEX_POINT('',#49941);
#10321=VERTEX_POINT('',#50073);
#10322=VERTEX_POINT('',#50269);
#10323=VERTEX_POINT('',#50270);
#10324=VERTEX_POINT('',#50272);
#10325=VERTEX_POINT('',#50351);
#10326=VERTEX_POINT('',#50432);
#10327=VERTEX_POINT('',#50433);
#10328=VERTEX_POINT('',#50435);
#10329=VERTEX_POINT('',#50566);
#10330=VERTEX_POINT('',#50698);
#10331=VERTEX_POINT('',#50699);
#10332=VERTEX_POINT('',#50701);
#10333=VERTEX_POINT('',#50899);
#10334=VERTEX_POINT('',#50979);
#10335=VERTEX_POINT('',#50980);
#10336=VERTEX_POINT('',#50982);
#10337=VERTEX_POINT('',#51180);
#10338=VERTEX_POINT('',#51312);
#10339=VERTEX_POINT('',#51313);
#10340=VERTEX_POINT('',#51315);
#10341=VERTEX_POINT('',#51394);
#10342=VERTEX_POINT('',#51593);
#10343=VERTEX_POINT('',#51594);
#10344=VERTEX_POINT('',#51596);
#10345=VERTEX_POINT('',#51603);
#10346=VERTEX_POINT('',#51609);
#10347=VERTEX_POINT('',#51611);
#10348=VERTEX_POINT('',#51678);
#10349=VERTEX_POINT('',#51679);
#10350=VERTEX_POINT('',#51681);
#10351=VERTEX_POINT('',#51690);
#10352=VERTEX_POINT('',#51696);
#10353=VERTEX_POINT('',#51698);
#10354=VERTEX_POINT('',#51766);
#10355=VERTEX_POINT('',#51767);
#10356=VERTEX_POINT('',#51769);
#10357=VERTEX_POINT('',#51900);
#10358=VERTEX_POINT('',#51917);
#10359=VERTEX_POINT('',#51918);
#10360=VERTEX_POINT('',#51920);
#10361=VERTEX_POINT('',#52118);
#10362=VERTEX_POINT('',#52250);
#10363=VERTEX_POINT('',#52251);
#10364=VERTEX_POINT('',#52253);
#10365=VERTEX_POINT('',#52332);
#10366=VERTEX_POINT('',#52531);
#10367=VERTEX_POINT('',#52532);
#10368=VERTEX_POINT('',#52534);
#10369=VERTEX_POINT('',#52668);
#10370=VERTEX_POINT('',#52867);
#10371=VERTEX_POINT('',#52868);
#10372=VERTEX_POINT('',#52870);
#10373=VERTEX_POINT('',#52949);
#10374=VERTEX_POINT('',#53029);
#10375=VERTEX_POINT('',#53030);
#10376=VERTEX_POINT('',#53032);
#10377=VERTEX_POINT('',#53167);
#10378=VERTEX_POINT('',#53299);
#10379=VERTEX_POINT('',#53300);
#10380=VERTEX_POINT('',#53302);
#10381=VERTEX_POINT('',#53494);
#10382=VERTEX_POINT('',#53574);
#10383=VERTEX_POINT('',#53575);
#10384=VERTEX_POINT('',#53577);
#10385=VERTEX_POINT('',#53772);
#10386=VERTEX_POINT('',#53908);
#10387=VERTEX_POINT('',#53909);
#10388=VERTEX_POINT('',#53911);
#10389=VERTEX_POINT('',#53990);
#10390=VERTEX_POINT('',#54070);
#10391=VERTEX_POINT('',#54071);
#10392=VERTEX_POINT('',#54073);
#10393=VERTEX_POINT('',#54205);
#10394=VERTEX_POINT('',#54337);
#10395=VERTEX_POINT('',#54338);
#10396=VERTEX_POINT('',#54340);
#10397=VERTEX_POINT('',#54535);
#10398=VERTEX_POINT('',#54615);
#10399=VERTEX_POINT('',#54616);
#10400=VERTEX_POINT('',#54618);
#10401=VERTEX_POINT('',#54816);
#10402=VERTEX_POINT('',#54948);
#10403=VERTEX_POINT('',#54949);
#10404=VERTEX_POINT('',#54951);
#10405=VERTEX_POINT('',#55030);
#10406=VERTEX_POINT('',#55113);
#10407=VERTEX_POINT('',#55114);
#10408=VERTEX_POINT('',#55116);
#10409=VERTEX_POINT('',#55250);
#10410=VERTEX_POINT('',#55382);
#10411=VERTEX_POINT('',#55383);
#10412=VERTEX_POINT('',#55385);
#10413=VERTEX_POINT('',#55464);
#10414=VERTEX_POINT('',#55663);
#10415=VERTEX_POINT('',#55664);
#10416=VERTEX_POINT('',#55666);
#10417=VERTEX_POINT('',#55800);
#10418=VERTEX_POINT('',#55996);
#10419=VERTEX_POINT('',#55997);
#10420=VERTEX_POINT('',#55999);
#10421=VERTEX_POINT('',#56075);
#10422=VERTEX_POINT('',#56155);
#10423=VERTEX_POINT('',#56156);
#10424=VERTEX_POINT('',#56158);
#10425=VERTEX_POINT('',#56289);
#10426=VERTEX_POINT('',#56425);
#10427=VERTEX_POINT('',#56426);
#10428=VERTEX_POINT('',#56428);
#10429=VERTEX_POINT('',#56507);
#10430=VERTEX_POINT('',#56706);
#10431=VERTEX_POINT('',#56707);
#10432=VERTEX_POINT('',#56709);
#10433=VERTEX_POINT('',#56841);
#10434=VERTEX_POINT('',#57037);
#10435=VERTEX_POINT('',#57038);
#10436=VERTEX_POINT('',#57040);
#10437=VERTEX_POINT('',#57119);
#10438=VERTEX_POINT('',#57200);
#10439=VERTEX_POINT('',#57201);
#10440=VERTEX_POINT('',#57203);
#10441=VERTEX_POINT('',#57334);
#10442=VERTEX_POINT('',#57466);
#10443=VERTEX_POINT('',#57467);
#10444=VERTEX_POINT('',#57469);
#10445=VERTEX_POINT('',#57667);
#10446=VERTEX_POINT('',#57747);
#10447=VERTEX_POINT('',#57748);
#10448=VERTEX_POINT('',#57750);
#10449=VERTEX_POINT('',#57948);
#10450=VERTEX_POINT('',#58080);
#10451=VERTEX_POINT('',#58081);
#10452=VERTEX_POINT('',#58083);
#10453=VERTEX_POINT('',#58162);
#10454=VERTEX_POINT('',#58361);
#10455=VERTEX_POINT('',#58362);
#10456=VERTEX_POINT('',#58364);
#10457=VERTEX_POINT('',#58371);
#10458=VERTEX_POINT('',#58377);
#10459=VERTEX_POINT('',#58379);
#10460=VERTEX_POINT('',#58446);
#10461=VERTEX_POINT('',#58447);
#10462=VERTEX_POINT('',#58449);
#10463=VERTEX_POINT('',#58458);
#10464=VERTEX_POINT('',#58464);
#10465=VERTEX_POINT('',#58466);
#10466=VERTEX_POINT('',#58534);
#10467=VERTEX_POINT('',#58535);
#10468=VERTEX_POINT('',#58537);
#10469=VERTEX_POINT('',#58668);
#10470=VERTEX_POINT('',#58685);
#10471=VERTEX_POINT('',#58686);
#10472=VERTEX_POINT('',#58688);
#10473=VERTEX_POINT('',#58886);
#10474=VERTEX_POINT('',#59018);
#10475=VERTEX_POINT('',#59019);
#10476=VERTEX_POINT('',#59021);
#10477=VERTEX_POINT('',#59100);
#10478=VERTEX_POINT('',#59299);
#10479=VERTEX_POINT('',#59300);
#10480=VERTEX_POINT('',#59302);
#10481=VERTEX_POINT('',#59436);
#10482=VERTEX_POINT('',#59635);
#10483=VERTEX_POINT('',#59636);
#10484=VERTEX_POINT('',#59638);
#10485=VERTEX_POINT('',#59717);
#10486=VERTEX_POINT('',#59797);
#10487=VERTEX_POINT('',#59798);
#10488=VERTEX_POINT('',#59800);
#10489=VERTEX_POINT('',#59935);
#10490=VERTEX_POINT('',#60067);
#10491=VERTEX_POINT('',#60068);
#10492=VERTEX_POINT('',#60070);
#10493=VERTEX_POINT('',#60262);
#10494=VERTEX_POINT('',#60342);
#10495=VERTEX_POINT('',#60343);
#10496=VERTEX_POINT('',#60345);
#10497=VERTEX_POINT('',#60540);
#10498=VERTEX_POINT('',#60676);
#10499=VERTEX_POINT('',#60677);
#10500=VERTEX_POINT('',#60679);
#10501=VERTEX_POINT('',#60758);
#10502=VERTEX_POINT('',#60838);
#10503=VERTEX_POINT('',#60839);
#10504=VERTEX_POINT('',#60841);
#10505=VERTEX_POINT('',#60973);
#10506=VERTEX_POINT('',#61105);
#10507=VERTEX_POINT('',#61106);
#10508=VERTEX_POINT('',#61108);
#10509=VERTEX_POINT('',#61303);
#10510=VERTEX_POINT('',#61383);
#10511=VERTEX_POINT('',#61384);
#10512=VERTEX_POINT('',#61386);
#10513=VERTEX_POINT('',#61584);
#10514=VERTEX_POINT('',#61716);
#10515=VERTEX_POINT('',#61717);
#10516=VERTEX_POINT('',#61719);
#10517=VERTEX_POINT('',#61798);
#10518=VERTEX_POINT('',#61881);
#10519=VERTEX_POINT('',#61882);
#10520=VERTEX_POINT('',#61884);
#10521=VERTEX_POINT('',#62018);
#10522=VERTEX_POINT('',#62150);
#10523=VERTEX_POINT('',#62151);
#10524=VERTEX_POINT('',#62153);
#10525=VERTEX_POINT('',#62232);
#10526=VERTEX_POINT('',#62431);
#10527=VERTEX_POINT('',#62432);
#10528=VERTEX_POINT('',#62434);
#10529=VERTEX_POINT('',#62568);
#10530=VERTEX_POINT('',#62764);
#10531=VERTEX_POINT('',#62765);
#10532=VERTEX_POINT('',#62767);
#10533=VERTEX_POINT('',#62843);
#10534=VERTEX_POINT('',#62923);
#10535=VERTEX_POINT('',#62924);
#10536=VERTEX_POINT('',#62926);
#10537=VERTEX_POINT('',#63057);
#10538=VERTEX_POINT('',#63193);
#10539=VERTEX_POINT('',#63194);
#10540=VERTEX_POINT('',#63196);
#10541=VERTEX_POINT('',#63275);
#10542=VERTEX_POINT('',#63474);
#10543=VERTEX_POINT('',#63475);
#10544=VERTEX_POINT('',#63477);
#10545=VERTEX_POINT('',#63609);
#10546=VERTEX_POINT('',#63805);
#10547=VERTEX_POINT('',#63806);
#10548=VERTEX_POINT('',#63808);
#10549=VERTEX_POINT('',#63887);
#10550=VERTEX_POINT('',#63968);
#10551=VERTEX_POINT('',#63969);
#10552=VERTEX_POINT('',#63971);
#10553=VERTEX_POINT('',#64102);
#10554=VERTEX_POINT('',#64234);
#10555=VERTEX_POINT('',#64235);
#10556=VERTEX_POINT('',#64237);
#10557=VERTEX_POINT('',#64435);
#10558=VERTEX_POINT('',#64515);
#10559=VERTEX_POINT('',#64516);
#10560=VERTEX_POINT('',#64518);
#10561=VERTEX_POINT('',#64716);
#10562=VERTEX_POINT('',#64848);
#10563=VERTEX_POINT('',#64849);
#10564=VERTEX_POINT('',#64851);
#10565=VERTEX_POINT('',#64930);
#10566=VERTEX_POINT('',#65129);
#10567=VERTEX_POINT('',#65130);
#10568=VERTEX_POINT('',#65132);
#10569=VERTEX_POINT('',#65139);
#10570=VERTEX_POINT('',#65145);
#10571=VERTEX_POINT('',#65147);
#10572=VERTEX_POINT('',#65214);
#10573=VERTEX_POINT('',#65215);
#10574=VERTEX_POINT('',#65217);
#10575=VERTEX_POINT('',#65256);
#10576=VERTEX_POINT('',#65258);
#10577=VERTEX_POINT('',#65291);
#10578=VERTEX_POINT('',#65292);
#10579=VERTEX_POINT('',#65294);
#10580=VERTEX_POINT('',#65362);
#10581=VERTEX_POINT('',#65591);
#10582=VERTEX_POINT('',#65592);
#10583=VERTEX_POINT('',#65594);
#10584=VERTEX_POINT('',#65809);
#10585=VERTEX_POINT('',#66044);
#10586=VERTEX_POINT('',#66045);
#10587=VERTEX_POINT('',#66047);
#10588=VERTEX_POINT('',#66064);
#10589=VERTEX_POINT('',#66065);
#10590=VERTEX_POINT('',#66067);
#10591=VERTEX_POINT('',#66084);
#10592=VERTEX_POINT('',#66085);
#10593=VERTEX_POINT('',#66087);
#10594=VERTEX_POINT('',#66358);
#10595=VERTEX_POINT('',#66359);
#10596=VERTEX_POINT('',#66361);
#10597=VERTEX_POINT('',#66595);
#10598=VERTEX_POINT('',#66811);
#10599=VERTEX_POINT('',#66812);
#10600=VERTEX_POINT('',#66814);
#10601=VERTEX_POINT('',#66853);
#10602=VERTEX_POINT('',#66855);
#10603=VERTEX_POINT('',#66888);
#10604=VERTEX_POINT('',#66889);
#10605=VERTEX_POINT('',#66891);
#10606=VERTEX_POINT('',#66918);
#10607=VERTEX_POINT('',#67037);
#10608=VERTEX_POINT('',#67039);
#10609=VERTEX_POINT('',#67218);
#10610=VERTEX_POINT('',#67219);
#10611=VERTEX_POINT('',#67688);
#10612=VERTEX_POINT('',#67689);
#10613=VERTEX_POINT('',#67691);
#10614=VERTEX_POINT('',#67906);
#10615=VERTEX_POINT('',#68144);
#10616=VERTEX_POINT('',#68145);
#10617=VERTEX_POINT('',#68147);
#10618=VERTEX_POINT('',#68402);
#10619=VERTEX_POINT('',#68403);
#10620=VERTEX_POINT('',#68405);
#10621=VERTEX_POINT('',#68601);
#10622=VERTEX_POINT('',#68849);
#10623=VERTEX_POINT('',#68850);
#10624=VERTEX_POINT('',#69359);
#10625=VERTEX_POINT('',#69360);
#10626=VERTEX_POINT('',#69362);
#10627=VERTEX_POINT('',#69629);
#10628=VERTEX_POINT('',#69865);
#10629=VERTEX_POINT('',#69866);
#10630=VERTEX_POINT('',#70341);
#10631=VERTEX_POINT('',#70342);
#10632=VERTEX_POINT('',#70344);
#10633=VERTEX_POINT('',#70577);
#10634=VERTEX_POINT('',#70825);
#10635=VERTEX_POINT('',#70826);
#10636=VERTEX_POINT('',#70828);
#10637=VERTEX_POINT('',#71117);
#10638=VERTEX_POINT('',#71118);
#10639=VERTEX_POINT('',#71120);
#10640=VERTEX_POINT('',#71322);
#10641=VERTEX_POINT('',#71553);
#10642=VERTEX_POINT('',#71554);
#10643=VERTEX_POINT('',#71776);
#10644=VERTEX_POINT('',#71964);
#10645=VERTEX_POINT('',#71965);
#10646=VERTEX_POINT('',#71967);
#10647=VERTEX_POINT('',#72214);
#10648=VERTEX_POINT('',#72234);
#10649=VERTEX_POINT('',#72235);
#10650=VERTEX_POINT('',#72744);
#10651=VERTEX_POINT('',#72745);
#10652=VERTEX_POINT('',#72747);
#10653=VERTEX_POINT('',#73011);
#10654=VERTEX_POINT('',#73247);
#10655=VERTEX_POINT('',#73248);
#10656=VERTEX_POINT('',#73250);
#10657=VERTEX_POINT('',#73511);
#10658=VERTEX_POINT('',#73512);
#10659=VERTEX_POINT('',#73514);
#10660=VERTEX_POINT('',#73714);
#10661=VERTEX_POINT('',#73945);
#10662=VERTEX_POINT('',#73946);
#10663=VERTEX_POINT('',#74184);
#10664=VERTEX_POINT('',#74368);
#10665=VERTEX_POINT('',#74369);
#10666=VERTEX_POINT('',#74371);
#10667=VERTEX_POINT('',#74628);
#10668=VERTEX_POINT('',#74662);
#10669=VERTEX_POINT('',#74663);
#10670=VERTEX_POINT('',#75136);
#10671=VERTEX_POINT('',#75137);
#10672=VERTEX_POINT('',#75139);
#10673=VERTEX_POINT('',#75380);
#10674=VERTEX_POINT('',#75622);
#10675=VERTEX_POINT('',#75623);
#10676=VERTEX_POINT('',#76122);
#10677=VERTEX_POINT('',#76123);
#10678=VERTEX_POINT('',#76125);
#10679=VERTEX_POINT('',#76370);
#10680=VERTEX_POINT('',#76636);
#10681=VERTEX_POINT('',#76637);
#10682=VERTEX_POINT('',#76869);
#10683=VERTEX_POINT('',#77056);
#10684=VERTEX_POINT('',#77057);
#10685=VERTEX_POINT('',#77059);
#10686=VERTEX_POINT('',#77296);
#10687=VERTEX_POINT('',#77314);
#10688=VERTEX_POINT('',#77315);
#10689=VERTEX_POINT('',#77776);
#10690=VERTEX_POINT('',#77777);
#10691=VERTEX_POINT('',#77779);
#10692=VERTEX_POINT('',#77886);
#10693=VERTEX_POINT('',#78049);
#10694=VERTEX_POINT('',#78050);
#10695=VERTEX_POINT('',#78052);
#10696=VERTEX_POINT('',#78079);
#10697=VERTEX_POINT('',#78198);
#10698=VERTEX_POINT('',#78200);
#10699=VERTEX_POINT('',#78379);
#10700=VERTEX_POINT('',#78380);
#10701=VERTEX_POINT('',#78843);
#10702=VERTEX_POINT('',#78844);
#10703=VERTEX_POINT('',#78846);
#10704=VERTEX_POINT('',#79061);
#10705=VERTEX_POINT('',#79301);
#10706=VERTEX_POINT('',#79302);
#10707=VERTEX_POINT('',#79304);
#10708=VERTEX_POINT('',#79557);
#10709=VERTEX_POINT('',#79558);
#10710=VERTEX_POINT('',#79560);
#10711=VERTEX_POINT('',#79756);
#10712=VERTEX_POINT('',#80002);
#10713=VERTEX_POINT('',#80003);
#10714=VERTEX_POINT('',#80512);
#10715=VERTEX_POINT('',#80513);
#10716=VERTEX_POINT('',#80515);
#10717=VERTEX_POINT('',#80782);
#10718=VERTEX_POINT('',#81016);
#10719=VERTEX_POINT('',#81017);
#10720=VERTEX_POINT('',#81526);
#10721=VERTEX_POINT('',#81527);
#10722=VERTEX_POINT('',#81529);
#10723=VERTEX_POINT('',#81752);
#10724=VERTEX_POINT('',#82000);
#10725=VERTEX_POINT('',#82001);
#10726=VERTEX_POINT('',#82003);
#10727=VERTEX_POINT('',#82292);
#10728=VERTEX_POINT('',#82293);
#10729=VERTEX_POINT('',#82295);
#10730=VERTEX_POINT('',#82497);
#10731=VERTEX_POINT('',#82724);
#10732=VERTEX_POINT('',#82725);
#10733=VERTEX_POINT('',#82947);
#10734=VERTEX_POINT('',#83135);
#10735=VERTEX_POINT('',#83136);
#10736=VERTEX_POINT('',#83138);
#10737=VERTEX_POINT('',#83389);
#10738=VERTEX_POINT('',#83409);
#10739=VERTEX_POINT('',#83410);
#10740=VERTEX_POINT('',#83901);
#10741=VERTEX_POINT('',#83902);
#10742=VERTEX_POINT('',#83904);
#10743=VERTEX_POINT('',#84166);
#10744=VERTEX_POINT('',#84402);
#10745=VERTEX_POINT('',#84403);
#10746=VERTEX_POINT('',#84405);
#10747=VERTEX_POINT('',#84658);
#10748=VERTEX_POINT('',#84659);
#10749=VERTEX_POINT('',#84661);
#10750=VERTEX_POINT('',#84859);
#10751=VERTEX_POINT('',#85090);
#10752=VERTEX_POINT('',#85091);
#10753=VERTEX_POINT('',#85329);
#10754=VERTEX_POINT('',#85513);
#10755=VERTEX_POINT('',#85514);
#10756=VERTEX_POINT('',#85516);
#10757=VERTEX_POINT('',#85775);
#10758=VERTEX_POINT('',#85809);
#10759=VERTEX_POINT('',#85810);
#10760=VERTEX_POINT('',#86287);
#10761=VERTEX_POINT('',#86288);
#10762=VERTEX_POINT('',#86290);
#10763=VERTEX_POINT('',#86575);
#10764=VERTEX_POINT('',#86817);
#10765=VERTEX_POINT('',#86818);
#10766=VERTEX_POINT('',#87313);
#10767=VERTEX_POINT('',#87314);
#10768=VERTEX_POINT('',#87316);
#10769=VERTEX_POINT('',#87557);
#10770=VERTEX_POINT('',#87847);
#10771=VERTEX_POINT('',#87848);
#10772=VERTEX_POINT('',#88080);
#10773=VERTEX_POINT('',#88267);
#10774=VERTEX_POINT('',#88268);
#10775=VERTEX_POINT('',#88270);
#10776=VERTEX_POINT('',#88509);
#10777=VERTEX_POINT('',#88527);
#10778=VERTEX_POINT('',#88528);
#10779=VERTEX_POINT('',#88993);
#10780=VERTEX_POINT('',#88994);
#10781=VERTEX_POINT('',#88996);
#10782=VERTEX_POINT('',#89103);
#10783=VERTEX_POINT('',#89266);
#10784=VERTEX_POINT('',#89267);
#10785=VERTEX_POINT('',#89269);
#10786=VERTEX_POINT('',#89296);
#10787=VERTEX_POINT('',#89415);
#10788=VERTEX_POINT('',#89417);
#10789=VERTEX_POINT('',#89596);
#10790=VERTEX_POINT('',#89597);
#10791=VERTEX_POINT('',#90058);
#10792=VERTEX_POINT('',#90059);
#10793=VERTEX_POINT('',#90061);
#10794=VERTEX_POINT('',#90276);
#10795=VERTEX_POINT('',#90514);
#10796=VERTEX_POINT('',#90515);
#10797=VERTEX_POINT('',#90517);
#10798=VERTEX_POINT('',#90764);
#10799=VERTEX_POINT('',#90765);
#10800=VERTEX_POINT('',#90767);
#10801=VERTEX_POINT('',#90963);
#10802=VERTEX_POINT('',#91209);
#10803=VERTEX_POINT('',#91210);
#10804=VERTEX_POINT('',#91731);
#10805=VERTEX_POINT('',#91732);
#10806=VERTEX_POINT('',#91734);
#10807=VERTEX_POINT('',#92001);
#10808=VERTEX_POINT('',#92235);
#10809=VERTEX_POINT('',#92236);
#10810=VERTEX_POINT('',#92701);
#10811=VERTEX_POINT('',#92702);
#10812=VERTEX_POINT('',#92704);
#10813=VERTEX_POINT('',#92927);
#10814=VERTEX_POINT('',#93175);
#10815=VERTEX_POINT('',#93176);
#10816=VERTEX_POINT('',#93178);
#10817=VERTEX_POINT('',#93467);
#10818=VERTEX_POINT('',#93468);
#10819=VERTEX_POINT('',#93470);
#10820=VERTEX_POINT('',#93672);
#10821=VERTEX_POINT('',#93899);
#10822=VERTEX_POINT('',#93900);
#10823=VERTEX_POINT('',#94122);
#10824=VERTEX_POINT('',#94310);
#10825=VERTEX_POINT('',#94311);
#10826=VERTEX_POINT('',#94313);
#10827=VERTEX_POINT('',#94558);
#10828=VERTEX_POINT('',#94578);
#10829=VERTEX_POINT('',#94579);
#10830=VERTEX_POINT('',#95072);
#10831=VERTEX_POINT('',#95073);
#10832=VERTEX_POINT('',#95075);
#10833=VERTEX_POINT('',#95337);
#10834=VERTEX_POINT('',#95573);
#10835=VERTEX_POINT('',#95574);
#10836=VERTEX_POINT('',#95576);
#10837=VERTEX_POINT('',#95837);
#10838=VERTEX_POINT('',#95838);
#10839=VERTEX_POINT('',#95840);
#10840=VERTEX_POINT('',#96040);
#10841=VERTEX_POINT('',#96271);
#10842=VERTEX_POINT('',#96272);
#10843=VERTEX_POINT('',#96508);
#10844=VERTEX_POINT('',#96692);
#10845=VERTEX_POINT('',#96693);
#10846=VERTEX_POINT('',#96695);
#10847=VERTEX_POINT('',#96952);
#10848=VERTEX_POINT('',#96986);
#10849=VERTEX_POINT('',#96987);
#10850=VERTEX_POINT('',#97464);
#10851=VERTEX_POINT('',#97465);
#10852=VERTEX_POINT('',#97467);
#10853=VERTEX_POINT('',#97708);
#10854=VERTEX_POINT('',#97950);
#10855=VERTEX_POINT('',#97951);
#10856=VERTEX_POINT('',#98446);
#10857=VERTEX_POINT('',#98447);
#10858=VERTEX_POINT('',#98449);
#10859=VERTEX_POINT('',#98692);
#10860=VERTEX_POINT('',#98960);
#10861=VERTEX_POINT('',#98961);
#10862=VERTEX_POINT('',#99193);
#10863=VERTEX_POINT('',#99380);
#10864=VERTEX_POINT('',#99381);
#10865=VERTEX_POINT('',#99383);
#10866=VERTEX_POINT('',#99624);
#10867=VERTEX_POINT('',#99642);
#10868=VERTEX_POINT('',#99643);
#10869=VERTEX_POINT('',#100104);
#10870=VERTEX_POINT('',#100105);
#10871=VERTEX_POINT('',#100107);
#10872=VERTEX_POINT('',#100214);
#10873=VERTEX_POINT('',#100377);
#10874=VERTEX_POINT('',#100378);
#10875=VERTEX_POINT('',#100380);
#10876=VERTEX_POINT('',#100407);
#10877=VERTEX_POINT('',#100526);
#10878=VERTEX_POINT('',#100528);
#10879=VERTEX_POINT('',#100707);
#10880=VERTEX_POINT('',#100708);
#10881=VERTEX_POINT('',#101177);
#10882=VERTEX_POINT('',#101178);
#10883=VERTEX_POINT('',#101180);
#10884=VERTEX_POINT('',#101395);
#10885=VERTEX_POINT('',#101635);
#10886=VERTEX_POINT('',#101636);
#10887=VERTEX_POINT('',#101638);
#10888=VERTEX_POINT('',#101889);
#10889=VERTEX_POINT('',#101890);
#10890=VERTEX_POINT('',#101892);
#10891=VERTEX_POINT('',#102088);
#10892=VERTEX_POINT('',#102334);
#10893=VERTEX_POINT('',#102335);
#10894=VERTEX_POINT('',#102842);
#10895=VERTEX_POINT('',#102843);
#10896=VERTEX_POINT('',#102845);
#10897=VERTEX_POINT('',#103112);
#10898=VERTEX_POINT('',#103346);
#10899=VERTEX_POINT('',#103347);
#10900=VERTEX_POINT('',#103868);
#10901=VERTEX_POINT('',#103869);
#10902=VERTEX_POINT('',#103871);
#10903=VERTEX_POINT('',#104102);
#10904=VERTEX_POINT('',#104352);
#10905=VERTEX_POINT('',#104353);
#10906=VERTEX_POINT('',#104355);
#10907=VERTEX_POINT('',#104646);
#10908=VERTEX_POINT('',#104647);
#10909=VERTEX_POINT('',#104649);
#10910=VERTEX_POINT('',#104851);
#10911=VERTEX_POINT('',#105082);
#10912=VERTEX_POINT('',#105083);
#10913=VERTEX_POINT('',#105305);
#10914=VERTEX_POINT('',#105493);
#10915=VERTEX_POINT('',#105494);
#10916=VERTEX_POINT('',#105496);
#10917=VERTEX_POINT('',#105737);
#10918=VERTEX_POINT('',#105757);
#10919=VERTEX_POINT('',#105758);
#10920=VERTEX_POINT('',#106249);
#10921=VERTEX_POINT('',#106250);
#10922=VERTEX_POINT('',#106252);
#10923=VERTEX_POINT('',#106518);
#10924=VERTEX_POINT('',#106802);
#10925=VERTEX_POINT('',#106803);
#10926=VERTEX_POINT('',#106805);
#10927=VERTEX_POINT('',#107062);
#10928=VERTEX_POINT('',#107063);
#10929=VERTEX_POINT('',#107065);
#10930=VERTEX_POINT('',#107263);
#10931=VERTEX_POINT('',#107494);
#10932=VERTEX_POINT('',#107495);
#10933=VERTEX_POINT('',#107733);
#10934=VERTEX_POINT('',#107917);
#10935=VERTEX_POINT('',#107918);
#10936=VERTEX_POINT('',#107920);
#10937=VERTEX_POINT('',#108179);
#10938=VERTEX_POINT('',#108213);
#10939=VERTEX_POINT('',#108214);
#10940=VERTEX_POINT('',#108687);
#10941=VERTEX_POINT('',#108688);
#10942=VERTEX_POINT('',#108690);
#10943=VERTEX_POINT('',#108931);
#10944=VERTEX_POINT('',#109165);
#10945=VERTEX_POINT('',#109166);
#10946=VERTEX_POINT('',#109661);
#10947=VERTEX_POINT('',#109662);
#10948=VERTEX_POINT('',#109664);
#10949=VERTEX_POINT('',#109911);
#10950=VERTEX_POINT('',#110185);
#10951=VERTEX_POINT('',#110186);
#10952=VERTEX_POINT('',#110418);
#10953=VERTEX_POINT('',#110605);
#10954=VERTEX_POINT('',#110606);
#10955=VERTEX_POINT('',#110608);
#10956=VERTEX_POINT('',#110847);
#10957=VERTEX_POINT('',#110865);
#10958=VERTEX_POINT('',#110866);
#10959=VERTEX_POINT('',#111327);
#10960=VERTEX_POINT('',#111328);
#10961=VERTEX_POINT('',#111330);
#10962=VERTEX_POINT('',#111437);
#10963=VERTEX_POINT('',#111600);
#10964=VERTEX_POINT('',#111838);
#10965=VERTEX_POINT('',#112075);
#10966=VERTEX_POINT('',#112315);
#10967=VERTEX_POINT('',#112552);
#10968=VERTEX_POINT('',#112792);
#10969=VERTEX_POINT('',#113029);
#10970=VERTEX_POINT('',#113259);
#10971=VERTEX_POINT('',#113496);
#10972=VERTEX_POINT('',#113724);
#10973=VERTEX_POINT('',#113845);
#10974=VERTEX_POINT('',#114062);
#10975=VERTEX_POINT('',#114077);
#10976=VERTEX_POINT('',#114157);
#10977=VERTEX_POINT('',#114172);
#10978=VERTEX_POINT('',#114252);
#10979=VERTEX_POINT('',#114267);
#10980=VERTEX_POINT('',#114347);
#10981=VERTEX_POINT('',#114362);
#10982=VERTEX_POINT('',#114442);
#10983=VERTEX_POINT('',#114537);
#10984=VERTEX_POINT('',#114778);
#10985=VERTEX_POINT('',#114873);
#10986=VERTEX_POINT('',#115114);
#10987=VERTEX_POINT('',#115116);
#10988=VERTEX_POINT('',#115121);
#10989=VERTEX_POINT('',#115122);
#10990=VERTEX_POINT('',#115124);
#10991=VERTEX_POINT('',#115126);
#10992=VERTEX_POINT('',#115130);
#10993=VERTEX_POINT('',#115132);
#10994=VERTEX_POINT('',#115134);
#10995=VERTEX_POINT('',#115138);
#10996=VERTEX_POINT('',#115140);
#10997=VERTEX_POINT('',#115145);
#10998=VERTEX_POINT('',#115146);
#10999=VERTEX_POINT('',#115148);
#11000=VERTEX_POINT('',#115150);
#11001=VERTEX_POINT('',#115154);
#11002=VERTEX_POINT('',#115155);
#11003=VERTEX_POINT('',#115158);
#11004=VERTEX_POINT('',#115162);
#11005=VERTEX_POINT('',#115164);
#11006=VERTEX_POINT('',#115169);
#11007=VERTEX_POINT('',#115171);
#11008=VERTEX_POINT('',#115175);
#11009=VERTEX_POINT('',#115177);
#11010=VERTEX_POINT('',#115179);
#11011=VERTEX_POINT('',#115184);
#11012=VERTEX_POINT('',#115188);
#11013=VERTEX_POINT('',#115190);
#11014=VERTEX_POINT('',#115192);
#11015=VERTEX_POINT('',#115194);
#11016=VERTEX_POINT('',#115196);
#11017=VERTEX_POINT('',#115198);
#11018=VERTEX_POINT('',#115200);
#11019=VERTEX_POINT('',#115202);
#11020=VERTEX_POINT('',#115204);
#11021=VERTEX_POINT('',#115206);
#11022=VERTEX_POINT('',#115208);
#11023=VERTEX_POINT('',#115210);
#11024=VERTEX_POINT('',#115212);
#11025=VERTEX_POINT('',#115214);
#11026=VERTEX_POINT('',#115216);
#11027=VERTEX_POINT('',#115218);
#11028=VERTEX_POINT('',#115220);
#11029=VERTEX_POINT('',#115222);
#11030=VERTEX_POINT('',#115224);
#11031=VERTEX_POINT('',#115226);
#11032=VERTEX_POINT('',#115228);
#11033=VERTEX_POINT('',#115230);
#11034=VERTEX_POINT('',#115232);
#11035=VERTEX_POINT('',#115234);
#11036=VERTEX_POINT('',#115236);
#11037=VERTEX_POINT('',#115238);
#11038=VERTEX_POINT('',#115240);
#11039=VERTEX_POINT('',#115243);
#11040=VERTEX_POINT('',#115245);
#11041=VERTEX_POINT('',#124043);
#11042=VERTEX_POINT('',#124044);
#11043=VERTEX_POINT('',#124046);
#11044=VERTEX_POINT('',#124048);
#11045=VERTEX_POINT('',#124052);
#11046=VERTEX_POINT('',#124054);
#11047=VERTEX_POINT('',#124058);
#11048=VERTEX_POINT('',#124060);
#11049=VERTEX_POINT('',#124064);
#11050=VERTEX_POINT('',#124066);
#11051=VERTEX_POINT('',#124070);
#11052=VERTEX_POINT('',#124072);
#11053=VERTEX_POINT('',#124076);
#11054=VERTEX_POINT('',#124078);
#11055=VERTEX_POINT('',#124085);
#11056=VERTEX_POINT('',#124087);
#11057=VERTEX_POINT('',#124092);
#11058=VERTEX_POINT('',#124093);
#11059=VERTEX_POINT('',#124095);
#11060=VERTEX_POINT('',#124097);
#11061=VERTEX_POINT('',#124101);
#11062=VERTEX_POINT('',#124103);
#11063=VERTEX_POINT('',#124107);
#11064=VERTEX_POINT('',#124109);
#11065=VERTEX_POINT('',#124119);
#11066=VERTEX_POINT('',#124121);
#11067=VERTEX_POINT('',#124124);
#11068=VERTEX_POINT('',#124125);
#11069=VERTEX_POINT('',#124127);
#11070=VERTEX_POINT('',#124129);
#11071=VERTEX_POINT('',#124133);
#11072=VERTEX_POINT('',#124135);
#11073=VERTEX_POINT('',#124139);
#11074=VERTEX_POINT('',#124141);
#11075=VERTEX_POINT('',#124145);
#11076=VERTEX_POINT('',#124147);
#11077=VERTEX_POINT('',#124151);
#11078=VERTEX_POINT('',#124153);
#11079=VERTEX_POINT('',#124157);
#11080=VERTEX_POINT('',#124159);
#11081=VERTEX_POINT('',#124166);
#11082=VERTEX_POINT('',#124168);
#11083=VERTEX_POINT('',#124175);
#11084=VERTEX_POINT('',#124181);
#11085=VERTEX_POINT('',#124186);
#11086=VERTEX_POINT('',#124187);
#11087=VERTEX_POINT('',#124189);
#11088=VERTEX_POINT('',#124191);
#11089=VERTEX_POINT('',#124195);
#11090=VERTEX_POINT('',#124197);
#11091=VERTEX_POINT('',#124201);
#11092=VERTEX_POINT('',#124203);
#11093=VERTEX_POINT('',#124213);
#11094=VERTEX_POINT('',#124215);
#11095=VERTEX_POINT('',#124218);
#11096=VERTEX_POINT('',#124219);
#11097=VERTEX_POINT('',#124221);
#11098=VERTEX_POINT('',#124223);
#11099=VERTEX_POINT('',#124227);
#11100=VERTEX_POINT('',#124229);
#11101=VERTEX_POINT('',#124233);
#11102=VERTEX_POINT('',#124235);
#11103=VERTEX_POINT('',#124239);
#11104=VERTEX_POINT('',#124241);
#11105=VERTEX_POINT('',#124245);
#11106=VERTEX_POINT('',#124247);
#11107=VERTEX_POINT('',#124251);
#11108=VERTEX_POINT('',#124253);
#11109=VERTEX_POINT('',#124260);
#11110=VERTEX_POINT('',#124262);
#11111=VERTEX_POINT('',#124267);
#11112=VERTEX_POINT('',#124268);
#11113=VERTEX_POINT('',#124270);
#11114=VERTEX_POINT('',#124272);
#11115=VERTEX_POINT('',#124276);
#11116=VERTEX_POINT('',#124278);
#11117=VERTEX_POINT('',#124282);
#11118=VERTEX_POINT('',#124284);
#11119=VERTEX_POINT('',#124288);
#11120=VERTEX_POINT('',#124290);
#11121=VERTEX_POINT('',#124294);
#11122=VERTEX_POINT('',#124296);
#11123=VERTEX_POINT('',#124300);
#11124=VERTEX_POINT('',#124302);
#11125=VERTEX_POINT('',#124309);
#11126=VERTEX_POINT('',#124311);
#11127=VERTEX_POINT('',#124318);
#11128=VERTEX_POINT('',#124320);
#11129=VERTEX_POINT('',#124325);
#11130=VERTEX_POINT('',#124330);
#11131=VERTEX_POINT('',#124335);
#11132=VERTEX_POINT('',#124340);
#11133=VERTEX_POINT('',#124345);
#11134=VERTEX_POINT('',#124351);
#11135=VERTEX_POINT('',#124355);
#11136=VERTEX_POINT('',#124359);
#11137=VERTEX_POINT('',#124363);
#11138=VERTEX_POINT('',#124367);
#11139=VERTEX_POINT('',#124371);
#11140=VERTEX_POINT('',#124377);
#11141=VERTEX_POINT('',#124381);
#11142=VERTEX_POINT('',#124385);
#11143=VERTEX_POINT('',#124389);
#11144=VERTEX_POINT('',#124393);
#11145=VERTEX_POINT('',#124397);
#11146=VERTEX_POINT('',#124401);
#11147=VERTEX_POINT('',#124405);
#11148=VERTEX_POINT('',#124409);
#11149=VERTEX_POINT('',#124413);
#11150=VERTEX_POINT('',#124417);
#11151=VERTEX_POINT('',#124421);
#13279=EDGE_CURVE('',#10088,#10089,#6413,.T.);
#13280=EDGE_CURVE('',#10089,#10090,#247,.T.);
#13281=EDGE_CURVE('',#10091,#10090,#5700,.T.);
#13282=EDGE_CURVE('',#10088,#10091,#248,.T.);
#13283=EDGE_CURVE('',#10092,#10093,#6414,.T.);
#13284=EDGE_CURVE('',#10093,#10094,#249,.T.);
#13285=EDGE_CURVE('',#10094,#10089,#250,.T.);
#13286=EDGE_CURVE('',#10095,#10088,#251,.T.);
#13287=EDGE_CURVE('',#10092,#10095,#252,.T.);
#13288=EDGE_CURVE('',#10096,#10097,#6415,.T.);
#13289=EDGE_CURVE('',#10097,#10098,#253,.T.);
#13290=EDGE_CURVE('',#10098,#10093,#254,.T.);
#13291=EDGE_CURVE('',#10099,#10092,#255,.T.);
#13292=EDGE_CURVE('',#10096,#10099,#256,.T.);
#13293=EDGE_CURVE('',#10100,#10101,#6416,.T.);
#13294=EDGE_CURVE('',#10102,#10100,#257,.T.);
#13295=EDGE_CURVE('',#10103,#10102,#258,.T.);
#13296=EDGE_CURVE('',#10104,#10103,#5701,.T.);
#13297=EDGE_CURVE('',#10104,#10105,#259,.T.);
#13298=EDGE_CURVE('',#10105,#10101,#260,.T.);
#13299=EDGE_CURVE('',#10106,#10107,#6417,.T.);
#13300=EDGE_CURVE('',#10107,#10108,#261,.T.);
#13301=EDGE_CURVE('',#10109,#10108,#5702,.T.);
#13302=EDGE_CURVE('',#10106,#10109,#262,.T.);
#13303=EDGE_CURVE('',#10110,#10111,#6418,.T.);
#13304=EDGE_CURVE('',#10111,#10112,#263,.T.);
#13305=EDGE_CURVE('',#10112,#10107,#264,.T.);
#13306=EDGE_CURVE('',#10113,#10106,#265,.T.);
#13307=EDGE_CURVE('',#10110,#10113,#266,.T.);
#13308=EDGE_CURVE('',#10114,#10115,#6419,.T.);
#13309=EDGE_CURVE('',#10115,#10116,#267,.T.);
#13310=EDGE_CURVE('',#10116,#10111,#268,.T.);
#13311=EDGE_CURVE('',#10117,#10110,#269,.T.);
#13312=EDGE_CURVE('',#10114,#10117,#270,.T.);
#13313=EDGE_CURVE('',#10118,#10119,#6420,.T.);
#13314=EDGE_CURVE('',#10120,#10118,#271,.T.);
#13315=EDGE_CURVE('',#10121,#10120,#272,.T.);
#13316=EDGE_CURVE('',#10122,#10121,#5703,.T.);
#13317=EDGE_CURVE('',#10122,#10123,#273,.T.);
#13318=EDGE_CURVE('',#10123,#10119,#274,.T.);
#13319=EDGE_CURVE('',#10124,#10125,#6421,.T.);
#13320=EDGE_CURVE('',#10125,#10126,#275,.T.);
#13321=EDGE_CURVE('',#10126,#10127,#276,.T.);
#13322=EDGE_CURVE('',#10128,#10127,#5704,.T.);
#13323=EDGE_CURVE('',#10129,#10128,#277,.T.);
#13324=EDGE_CURVE('',#10124,#10129,#278,.T.);
#13325=EDGE_CURVE('',#10130,#10131,#6422,.T.);
#13326=EDGE_CURVE('',#10131,#10132,#279,.T.);
#13327=EDGE_CURVE('',#10132,#10125,#280,.T.);
#13328=EDGE_CURVE('',#10133,#10124,#281,.T.);
#13329=EDGE_CURVE('',#10130,#10133,#282,.T.);
#13330=EDGE_CURVE('',#10134,#10135,#6423,.T.);
#13331=EDGE_CURVE('',#10135,#10136,#283,.T.);
#13332=EDGE_CURVE('',#10136,#10131,#284,.T.);
#13333=EDGE_CURVE('',#10137,#10130,#285,.T.);
#13334=EDGE_CURVE('',#10134,#10137,#286,.T.);
#13335=EDGE_CURVE('',#10138,#10139,#6424,.T.);
#13336=EDGE_CURVE('',#10139,#10140,#287,.T.);
#13337=EDGE_CURVE('',#10140,#10135,#288,.T.);
#13338=EDGE_CURVE('',#10141,#10134,#289,.T.);
#13339=EDGE_CURVE('',#10138,#10141,#290,.T.);
#13340=EDGE_CURVE('',#10142,#10143,#6425,.T.);
#13341=EDGE_CURVE('',#10143,#10144,#291,.T.);
#13342=EDGE_CURVE('',#10144,#10139,#292,.T.);
#13343=EDGE_CURVE('',#10145,#10138,#293,.T.);
#13344=EDGE_CURVE('',#10142,#10145,#294,.T.);
#13345=EDGE_CURVE('',#10146,#10147,#6426,.T.);
#13346=EDGE_CURVE('',#10147,#10148,#295,.T.);
#13347=EDGE_CURVE('',#10148,#10143,#296,.T.);
#13348=EDGE_CURVE('',#10149,#10142,#297,.T.);
#13349=EDGE_CURVE('',#10146,#10149,#298,.T.);
#13350=EDGE_CURVE('',#10150,#10151,#6427,.T.);
#13351=EDGE_CURVE('',#10151,#10152,#299,.T.);
#13352=EDGE_CURVE('',#10152,#10147,#300,.T.);
#13353=EDGE_CURVE('',#10153,#10146,#301,.T.);
#13354=EDGE_CURVE('',#10150,#10153,#302,.T.);
#13355=EDGE_CURVE('',#10154,#10155,#6428,.T.);
#13356=EDGE_CURVE('',#10155,#10156,#303,.T.);
#13357=EDGE_CURVE('',#10156,#10151,#304,.T.);
#13358=EDGE_CURVE('',#10157,#10150,#305,.T.);
#13359=EDGE_CURVE('',#10154,#10157,#306,.T.);
#13360=EDGE_CURVE('',#10158,#10159,#6429,.T.);
#13361=EDGE_CURVE('',#10159,#10160,#307,.T.);
#13362=EDGE_CURVE('',#10160,#10155,#308,.T.);
#13363=EDGE_CURVE('',#10161,#10154,#309,.T.);
#13364=EDGE_CURVE('',#10158,#10161,#310,.T.);
#13365=EDGE_CURVE('',#10162,#10163,#6430,.T.);
#13366=EDGE_CURVE('',#10163,#10164,#311,.T.);
#13367=EDGE_CURVE('',#10164,#10159,#312,.T.);
#13368=EDGE_CURVE('',#10165,#10158,#313,.T.);
#13369=EDGE_CURVE('',#10162,#10165,#314,.T.);
#13370=EDGE_CURVE('',#10166,#10167,#6431,.T.);
#13371=EDGE_CURVE('',#10167,#10168,#315,.T.);
#13372=EDGE_CURVE('',#10168,#10163,#316,.T.);
#13373=EDGE_CURVE('',#10169,#10162,#317,.T.);
#13374=EDGE_CURVE('',#10166,#10169,#318,.T.);
#13375=EDGE_CURVE('',#10170,#10171,#6432,.T.);
#13376=EDGE_CURVE('',#10171,#10172,#319,.T.);
#13377=EDGE_CURVE('',#10172,#10167,#320,.T.);
#13378=EDGE_CURVE('',#10173,#10166,#321,.T.);
#13379=EDGE_CURVE('',#10170,#10173,#322,.T.);
#13380=EDGE_CURVE('',#10174,#10175,#6433,.T.);
#13381=EDGE_CURVE('',#10175,#10176,#323,.T.);
#13382=EDGE_CURVE('',#10176,#10171,#324,.T.);
#13383=EDGE_CURVE('',#10177,#10170,#325,.T.);
#13384=EDGE_CURVE('',#10174,#10177,#326,.T.);
#13385=EDGE_CURVE('',#10178,#10179,#6434,.T.);
#13386=EDGE_CURVE('',#10179,#10180,#327,.T.);
#13387=EDGE_CURVE('',#10180,#10175,#328,.T.);
#13388=EDGE_CURVE('',#10181,#10174,#329,.T.);
#13389=EDGE_CURVE('',#10178,#10181,#330,.T.);
#13390=EDGE_CURVE('',#10182,#10183,#6435,.T.);
#13391=EDGE_CURVE('',#10183,#10184,#331,.T.);
#13392=EDGE_CURVE('',#10184,#10179,#332,.T.);
#13393=EDGE_CURVE('',#10185,#10178,#333,.T.);
#13394=EDGE_CURVE('',#10182,#10185,#334,.T.);
#13395=EDGE_CURVE('',#10186,#10187,#6436,.T.);
#13396=EDGE_CURVE('',#10187,#10188,#335,.T.);
#13397=EDGE_CURVE('',#10188,#10183,#336,.T.);
#13398=EDGE_CURVE('',#10189,#10182,#337,.T.);
#13399=EDGE_CURVE('',#10186,#10189,#338,.T.);
#13400=EDGE_CURVE('',#10190,#10191,#6437,.T.);
#13401=EDGE_CURVE('',#10191,#10192,#339,.T.);
#13402=EDGE_CURVE('',#10192,#10187,#340,.T.);
#13403=EDGE_CURVE('',#10193,#10186,#341,.T.);
#13404=EDGE_CURVE('',#10190,#10193,#342,.T.);
#13405=EDGE_CURVE('',#10194,#10195,#6438,.T.);
#13406=EDGE_CURVE('',#10195,#10196,#343,.T.);
#13407=EDGE_CURVE('',#10196,#10191,#344,.T.);
#13408=EDGE_CURVE('',#10197,#10190,#345,.T.);
#13409=EDGE_CURVE('',#10194,#10197,#346,.T.);
#13410=EDGE_CURVE('',#10198,#10199,#6439,.T.);
#13411=EDGE_CURVE('',#10199,#10200,#347,.T.);
#13412=EDGE_CURVE('',#10200,#10195,#348,.T.);
#13413=EDGE_CURVE('',#10201,#10194,#349,.T.);
#13414=EDGE_CURVE('',#10198,#10201,#350,.T.);
#13415=EDGE_CURVE('',#10202,#10203,#6440,.T.);
#13416=EDGE_CURVE('',#10203,#10204,#351,.T.);
#13417=EDGE_CURVE('',#10204,#10199,#352,.T.);
#13418=EDGE_CURVE('',#10205,#10198,#353,.T.);
#13419=EDGE_CURVE('',#10202,#10205,#354,.T.);
#13420=EDGE_CURVE('',#10206,#10207,#6441,.T.);
#13421=EDGE_CURVE('',#10207,#10208,#355,.T.);
#13422=EDGE_CURVE('',#10208,#10203,#356,.T.);
#13423=EDGE_CURVE('',#10209,#10202,#357,.T.);
#13424=EDGE_CURVE('',#10206,#10209,#358,.T.);
#13425=EDGE_CURVE('',#10210,#10211,#6442,.T.);
#13426=EDGE_CURVE('',#10211,#10212,#359,.T.);
#13427=EDGE_CURVE('',#10212,#10207,#360,.T.);
#13428=EDGE_CURVE('',#10213,#10206,#361,.T.);
#13429=EDGE_CURVE('',#10210,#10213,#362,.T.);
#13430=EDGE_CURVE('',#10214,#10215,#6443,.T.);
#13431=EDGE_CURVE('',#10215,#10216,#363,.T.);
#13432=EDGE_CURVE('',#10216,#10211,#364,.T.);
#13433=EDGE_CURVE('',#10217,#10210,#365,.T.);
#13434=EDGE_CURVE('',#10214,#10217,#366,.T.);
#13435=EDGE_CURVE('',#10218,#10219,#6444,.T.);
#13436=EDGE_CURVE('',#10219,#10220,#367,.T.);
#13437=EDGE_CURVE('',#10220,#10215,#368,.T.);
#13438=EDGE_CURVE('',#10221,#10214,#369,.T.);
#13439=EDGE_CURVE('',#10218,#10221,#370,.T.);
#13440=EDGE_CURVE('',#10222,#10223,#6445,.T.);
#13441=EDGE_CURVE('',#10223,#10224,#371,.T.);
#13442=EDGE_CURVE('',#10224,#10219,#372,.T.);
#13443=EDGE_CURVE('',#10225,#10218,#373,.T.);
#13444=EDGE_CURVE('',#10222,#10225,#374,.T.);
#13445=EDGE_CURVE('',#10226,#10227,#6446,.T.);
#13446=EDGE_CURVE('',#10227,#10228,#375,.T.);
#13447=EDGE_CURVE('',#10228,#10223,#376,.T.);
#13448=EDGE_CURVE('',#10229,#10222,#377,.T.);
#13449=EDGE_CURVE('',#10226,#10229,#378,.T.);
#13450=EDGE_CURVE('',#10230,#10231,#6447,.T.);
#13451=EDGE_CURVE('',#10232,#10230,#379,.T.);
#13452=EDGE_CURVE('',#10233,#10232,#380,.T.);
#13453=EDGE_CURVE('',#10234,#10233,#5705,.T.);
#13454=EDGE_CURVE('',#10234,#10235,#381,.T.);
#13455=EDGE_CURVE('',#10235,#10231,#382,.T.);
#13456=EDGE_CURVE('',#10236,#10237,#6448,.T.);
#13457=EDGE_CURVE('',#10237,#10238,#383,.T.);
#13458=EDGE_CURVE('',#10238,#10239,#384,.T.);
#13459=EDGE_CURVE('',#10240,#10239,#5706,.T.);
#13460=EDGE_CURVE('',#10241,#10240,#385,.T.);
#13461=EDGE_CURVE('',#10236,#10241,#386,.T.);
#13462=EDGE_CURVE('',#10242,#10243,#6449,.T.);
#13463=EDGE_CURVE('',#10243,#10244,#387,.T.);
#13464=EDGE_CURVE('',#10244,#10237,#388,.T.);
#13465=EDGE_CURVE('',#10245,#10236,#389,.T.);
#13466=EDGE_CURVE('',#10242,#10245,#390,.T.);
#13467=EDGE_CURVE('',#10246,#10247,#6450,.T.);
#13468=EDGE_CURVE('',#10247,#10248,#391,.T.);
#13469=EDGE_CURVE('',#10248,#10243,#392,.T.);
#13470=EDGE_CURVE('',#10249,#10242,#393,.T.);
#13471=EDGE_CURVE('',#10246,#10249,#394,.T.);
#13472=EDGE_CURVE('',#10250,#10251,#6451,.T.);
#13473=EDGE_CURVE('',#10251,#10252,#395,.T.);
#13474=EDGE_CURVE('',#10252,#10247,#396,.T.);
#13475=EDGE_CURVE('',#10253,#10246,#397,.T.);
#13476=EDGE_CURVE('',#10250,#10253,#398,.T.);
#13477=EDGE_CURVE('',#10254,#10255,#6452,.T.);
#13478=EDGE_CURVE('',#10255,#10256,#399,.T.);
#13479=EDGE_CURVE('',#10256,#10251,#400,.T.);
#13480=EDGE_CURVE('',#10257,#10250,#401,.T.);
#13481=EDGE_CURVE('',#10254,#10257,#402,.T.);
#13482=EDGE_CURVE('',#10258,#10259,#6453,.T.);
#13483=EDGE_CURVE('',#10259,#10260,#403,.T.);
#13484=EDGE_CURVE('',#10260,#10255,#404,.T.);
#13485=EDGE_CURVE('',#10261,#10254,#405,.T.);
#13486=EDGE_CURVE('',#10258,#10261,#406,.T.);
#13487=EDGE_CURVE('',#10262,#10263,#6454,.T.);
#13488=EDGE_CURVE('',#10263,#10264,#407,.T.);
#13489=EDGE_CURVE('',#10264,#10259,#408,.T.);
#13490=EDGE_CURVE('',#10265,#10258,#409,.T.);
#13491=EDGE_CURVE('',#10262,#10265,#410,.T.);
#13492=EDGE_CURVE('',#10266,#10267,#6455,.T.);
#13493=EDGE_CURVE('',#10267,#10268,#411,.T.);
#13494=EDGE_CURVE('',#10268,#10263,#412,.T.);
#13495=EDGE_CURVE('',#10269,#10262,#413,.T.);
#13496=EDGE_CURVE('',#10266,#10269,#414,.T.);
#13497=EDGE_CURVE('',#10270,#10271,#6456,.T.);
#13498=EDGE_CURVE('',#10271,#10272,#415,.T.);
#13499=EDGE_CURVE('',#10272,#10267,#416,.T.);
#13500=EDGE_CURVE('',#10273,#10266,#417,.T.);
#13501=EDGE_CURVE('',#10270,#10273,#418,.T.);
#13502=EDGE_CURVE('',#10274,#10275,#6457,.T.);
#13503=EDGE_CURVE('',#10275,#10276,#419,.T.);
#13504=EDGE_CURVE('',#10276,#10271,#420,.T.);
#13505=EDGE_CURVE('',#10277,#10270,#421,.T.);
#13506=EDGE_CURVE('',#10274,#10277,#422,.T.);
#13507=EDGE_CURVE('',#10278,#10279,#6458,.T.);
#13508=EDGE_CURVE('',#10279,#10280,#423,.T.);
#13509=EDGE_CURVE('',#10280,#10275,#424,.T.);
#13510=EDGE_CURVE('',#10281,#10274,#425,.T.);
#13511=EDGE_CURVE('',#10278,#10281,#426,.T.);
#13512=EDGE_CURVE('',#10282,#10283,#6459,.T.);
#13513=EDGE_CURVE('',#10283,#10284,#427,.T.);
#13514=EDGE_CURVE('',#10284,#10279,#428,.T.);
#13515=EDGE_CURVE('',#10285,#10278,#429,.T.);
#13516=EDGE_CURVE('',#10282,#10285,#430,.T.);
#13517=EDGE_CURVE('',#10286,#10287,#6460,.T.);
#13518=EDGE_CURVE('',#10287,#10288,#431,.T.);
#13519=EDGE_CURVE('',#10288,#10283,#432,.T.);
#13520=EDGE_CURVE('',#10289,#10282,#433,.T.);
#13521=EDGE_CURVE('',#10286,#10289,#434,.T.);
#13522=EDGE_CURVE('',#10290,#10291,#6461,.T.);
#13523=EDGE_CURVE('',#10291,#10292,#435,.T.);
#13524=EDGE_CURVE('',#10292,#10287,#436,.T.);
#13525=EDGE_CURVE('',#10293,#10286,#437,.T.);
#13526=EDGE_CURVE('',#10290,#10293,#438,.T.);
#13527=EDGE_CURVE('',#10294,#10295,#6462,.T.);
#13528=EDGE_CURVE('',#10295,#10296,#439,.T.);
#13529=EDGE_CURVE('',#10296,#10291,#440,.T.);
#13530=EDGE_CURVE('',#10297,#10290,#441,.T.);
#13531=EDGE_CURVE('',#10294,#10297,#442,.T.);
#13532=EDGE_CURVE('',#10298,#10299,#6463,.T.);
#13533=EDGE_CURVE('',#10299,#10300,#443,.T.);
#13534=EDGE_CURVE('',#10300,#10295,#444,.T.);
#13535=EDGE_CURVE('',#10301,#10294,#445,.T.);
#13536=EDGE_CURVE('',#10298,#10301,#446,.T.);
#13537=EDGE_CURVE('',#10302,#10303,#6464,.T.);
#13538=EDGE_CURVE('',#10303,#10304,#447,.T.);
#13539=EDGE_CURVE('',#10304,#10299,#448,.T.);
#13540=EDGE_CURVE('',#10305,#10298,#449,.T.);
#13541=EDGE_CURVE('',#10302,#10305,#450,.T.);
#13542=EDGE_CURVE('',#10306,#10307,#6465,.T.);
#13543=EDGE_CURVE('',#10307,#10308,#451,.T.);
#13544=EDGE_CURVE('',#10308,#10303,#452,.T.);
#13545=EDGE_CURVE('',#10309,#10302,#453,.T.);
#13546=EDGE_CURVE('',#10306,#10309,#454,.T.);
#13547=EDGE_CURVE('',#10310,#10311,#6466,.T.);
#13548=EDGE_CURVE('',#10311,#10312,#455,.T.);
#13549=EDGE_CURVE('',#10312,#10307,#456,.T.);
#13550=EDGE_CURVE('',#10313,#10306,#457,.T.);
#13551=EDGE_CURVE('',#10310,#10313,#458,.T.);
#13552=EDGE_CURVE('',#10314,#10315,#6467,.T.);
#13553=EDGE_CURVE('',#10315,#10316,#459,.T.);
#13554=EDGE_CURVE('',#10316,#10311,#460,.T.);
#13555=EDGE_CURVE('',#10317,#10310,#461,.T.);
#13556=EDGE_CURVE('',#10314,#10317,#462,.T.);
#13557=EDGE_CURVE('',#10318,#10319,#6468,.T.);
#13558=EDGE_CURVE('',#10319,#10320,#463,.T.);
#13559=EDGE_CURVE('',#10320,#10315,#464,.T.);
#13560=EDGE_CURVE('',#10321,#10314,#465,.T.);
#13561=EDGE_CURVE('',#10318,#10321,#466,.T.);
#13562=EDGE_CURVE('',#10322,#10323,#6469,.T.);
#13563=EDGE_CURVE('',#10323,#10324,#467,.T.);
#13564=EDGE_CURVE('',#10324,#10319,#468,.T.);
#13565=EDGE_CURVE('',#10325,#10318,#469,.T.);
#13566=EDGE_CURVE('',#10322,#10325,#470,.T.);
#13567=EDGE_CURVE('',#10326,#10327,#6470,.T.);
#13568=EDGE_CURVE('',#10327,#10328,#471,.T.);
#13569=EDGE_CURVE('',#10328,#10323,#472,.T.);
#13570=EDGE_CURVE('',#10329,#10322,#473,.T.);
#13571=EDGE_CURVE('',#10326,#10329,#474,.T.);
#13572=EDGE_CURVE('',#10330,#10331,#6471,.T.);
#13573=EDGE_CURVE('',#10331,#10332,#475,.T.);
#13574=EDGE_CURVE('',#10332,#10327,#476,.T.);
#13575=EDGE_CURVE('',#10333,#10326,#477,.T.);
#13576=EDGE_CURVE('',#10330,#10333,#478,.T.);
#13577=EDGE_CURVE('',#10334,#10335,#6472,.T.);
#13578=EDGE_CURVE('',#10335,#10336,#479,.T.);
#13579=EDGE_CURVE('',#10336,#10331,#480,.T.);
#13580=EDGE_CURVE('',#10337,#10330,#481,.T.);
#13581=EDGE_CURVE('',#10334,#10337,#482,.T.);
#13582=EDGE_CURVE('',#10338,#10339,#6473,.T.);
#13583=EDGE_CURVE('',#10339,#10340,#483,.T.);
#13584=EDGE_CURVE('',#10340,#10335,#484,.T.);
#13585=EDGE_CURVE('',#10341,#10334,#485,.T.);
#13586=EDGE_CURVE('',#10338,#10341,#486,.T.);
#13587=EDGE_CURVE('',#10342,#10343,#6474,.T.);
#13588=EDGE_CURVE('',#10344,#10342,#487,.T.);
#13589=EDGE_CURVE('',#10345,#10344,#488,.T.);
#13590=EDGE_CURVE('',#10346,#10345,#5707,.T.);
#13591=EDGE_CURVE('',#10346,#10347,#489,.T.);
#13592=EDGE_CURVE('',#10347,#10343,#490,.T.);
#13593=EDGE_CURVE('',#10348,#10349,#6475,.T.);
#13594=EDGE_CURVE('',#10349,#10350,#491,.T.);
#13595=EDGE_CURVE('',#10350,#10351,#492,.T.);
#13596=EDGE_CURVE('',#10352,#10351,#5708,.T.);
#13597=EDGE_CURVE('',#10353,#10352,#493,.T.);
#13598=EDGE_CURVE('',#10348,#10353,#494,.T.);
#13599=EDGE_CURVE('',#10354,#10355,#6476,.T.);
#13600=EDGE_CURVE('',#10355,#10356,#495,.T.);
#13601=EDGE_CURVE('',#10356,#10349,#496,.T.);
#13602=EDGE_CURVE('',#10357,#10348,#497,.T.);
#13603=EDGE_CURVE('',#10354,#10357,#498,.T.);
#13604=EDGE_CURVE('',#10358,#10359,#6477,.T.);
#13605=EDGE_CURVE('',#10359,#10360,#499,.T.);
#13606=EDGE_CURVE('',#10360,#10355,#500,.T.);
#13607=EDGE_CURVE('',#10361,#10354,#501,.T.);
#13608=EDGE_CURVE('',#10358,#10361,#502,.T.);
#13609=EDGE_CURVE('',#10362,#10363,#6478,.T.);
#13610=EDGE_CURVE('',#10363,#10364,#503,.T.);
#13611=EDGE_CURVE('',#10364,#10359,#504,.T.);
#13612=EDGE_CURVE('',#10365,#10358,#505,.T.);
#13613=EDGE_CURVE('',#10362,#10365,#506,.T.);
#13614=EDGE_CURVE('',#10366,#10367,#6479,.T.);
#13615=EDGE_CURVE('',#10367,#10368,#507,.T.);
#13616=EDGE_CURVE('',#10368,#10363,#508,.T.);
#13617=EDGE_CURVE('',#10369,#10362,#509,.T.);
#13618=EDGE_CURVE('',#10366,#10369,#510,.T.);
#13619=EDGE_CURVE('',#10370,#10371,#6480,.T.);
#13620=EDGE_CURVE('',#10371,#10372,#511,.T.);
#13621=EDGE_CURVE('',#10372,#10367,#512,.T.);
#13622=EDGE_CURVE('',#10373,#10366,#513,.T.);
#13623=EDGE_CURVE('',#10370,#10373,#514,.T.);
#13624=EDGE_CURVE('',#10374,#10375,#6481,.T.);
#13625=EDGE_CURVE('',#10375,#10376,#515,.T.);
#13626=EDGE_CURVE('',#10376,#10371,#516,.T.);
#13627=EDGE_CURVE('',#10377,#10370,#517,.T.);
#13628=EDGE_CURVE('',#10374,#10377,#518,.T.);
#13629=EDGE_CURVE('',#10378,#10379,#6482,.T.);
#13630=EDGE_CURVE('',#10379,#10380,#519,.T.);
#13631=EDGE_CURVE('',#10380,#10375,#520,.T.);
#13632=EDGE_CURVE('',#10381,#10374,#521,.T.);
#13633=EDGE_CURVE('',#10378,#10381,#522,.T.);
#13634=EDGE_CURVE('',#10382,#10383,#6483,.T.);
#13635=EDGE_CURVE('',#10383,#10384,#523,.T.);
#13636=EDGE_CURVE('',#10384,#10379,#524,.T.);
#13637=EDGE_CURVE('',#10385,#10378,#525,.T.);
#13638=EDGE_CURVE('',#10382,#10385,#526,.T.);
#13639=EDGE_CURVE('',#10386,#10387,#6484,.T.);
#13640=EDGE_CURVE('',#10387,#10388,#527,.T.);
#13641=EDGE_CURVE('',#10388,#10383,#528,.T.);
#13642=EDGE_CURVE('',#10389,#10382,#529,.T.);
#13643=EDGE_CURVE('',#10386,#10389,#530,.T.);
#13644=EDGE_CURVE('',#10390,#10391,#6485,.T.);
#13645=EDGE_CURVE('',#10391,#10392,#531,.T.);
#13646=EDGE_CURVE('',#10392,#10387,#532,.T.);
#13647=EDGE_CURVE('',#10393,#10386,#533,.T.);
#13648=EDGE_CURVE('',#10390,#10393,#534,.T.);
#13649=EDGE_CURVE('',#10394,#10395,#6486,.T.);
#13650=EDGE_CURVE('',#10395,#10396,#535,.T.);
#13651=EDGE_CURVE('',#10396,#10391,#536,.T.);
#13652=EDGE_CURVE('',#10397,#10390,#537,.T.);
#13653=EDGE_CURVE('',#10394,#10397,#538,.T.);
#13654=EDGE_CURVE('',#10398,#10399,#6487,.T.);
#13655=EDGE_CURVE('',#10399,#10400,#539,.T.);
#13656=EDGE_CURVE('',#10400,#10395,#540,.T.);
#13657=EDGE_CURVE('',#10401,#10394,#541,.T.);
#13658=EDGE_CURVE('',#10398,#10401,#542,.T.);
#13659=EDGE_CURVE('',#10402,#10403,#6488,.T.);
#13660=EDGE_CURVE('',#10403,#10404,#543,.T.);
#13661=EDGE_CURVE('',#10404,#10399,#544,.T.);
#13662=EDGE_CURVE('',#10405,#10398,#545,.T.);
#13663=EDGE_CURVE('',#10402,#10405,#546,.T.);
#13664=EDGE_CURVE('',#10406,#10407,#6489,.T.);
#13665=EDGE_CURVE('',#10407,#10408,#547,.T.);
#13666=EDGE_CURVE('',#10408,#10403,#548,.T.);
#13667=EDGE_CURVE('',#10409,#10402,#549,.T.);
#13668=EDGE_CURVE('',#10406,#10409,#550,.T.);
#13669=EDGE_CURVE('',#10410,#10411,#6490,.T.);
#13670=EDGE_CURVE('',#10411,#10412,#551,.T.);
#13671=EDGE_CURVE('',#10412,#10407,#552,.T.);
#13672=EDGE_CURVE('',#10413,#10406,#553,.T.);
#13673=EDGE_CURVE('',#10410,#10413,#554,.T.);
#13674=EDGE_CURVE('',#10414,#10415,#6491,.T.);
#13675=EDGE_CURVE('',#10415,#10416,#555,.T.);
#13676=EDGE_CURVE('',#10416,#10411,#556,.T.);
#13677=EDGE_CURVE('',#10417,#10410,#557,.T.);
#13678=EDGE_CURVE('',#10414,#10417,#558,.T.);
#13679=EDGE_CURVE('',#10418,#10419,#6492,.T.);
#13680=EDGE_CURVE('',#10419,#10420,#559,.T.);
#13681=EDGE_CURVE('',#10420,#10415,#560,.T.);
#13682=EDGE_CURVE('',#10421,#10414,#561,.T.);
#13683=EDGE_CURVE('',#10418,#10421,#562,.T.);
#13684=EDGE_CURVE('',#10422,#10423,#6493,.T.);
#13685=EDGE_CURVE('',#10423,#10424,#563,.T.);
#13686=EDGE_CURVE('',#10424,#10419,#564,.T.);
#13687=EDGE_CURVE('',#10425,#10418,#565,.T.);
#13688=EDGE_CURVE('',#10422,#10425,#566,.T.);
#13689=EDGE_CURVE('',#10426,#10427,#6494,.T.);
#13690=EDGE_CURVE('',#10427,#10428,#567,.T.);
#13691=EDGE_CURVE('',#10428,#10423,#568,.T.);
#13692=EDGE_CURVE('',#10429,#10422,#569,.T.);
#13693=EDGE_CURVE('',#10426,#10429,#570,.T.);
#13694=EDGE_CURVE('',#10430,#10431,#6495,.T.);
#13695=EDGE_CURVE('',#10431,#10432,#571,.T.);
#13696=EDGE_CURVE('',#10432,#10427,#572,.T.);
#13697=EDGE_CURVE('',#10433,#10426,#573,.T.);
#13698=EDGE_CURVE('',#10430,#10433,#574,.T.);
#13699=EDGE_CURVE('',#10434,#10435,#6496,.T.);
#13700=EDGE_CURVE('',#10435,#10436,#575,.T.);
#13701=EDGE_CURVE('',#10436,#10431,#576,.T.);
#13702=EDGE_CURVE('',#10437,#10430,#577,.T.);
#13703=EDGE_CURVE('',#10434,#10437,#578,.T.);
#13704=EDGE_CURVE('',#10438,#10439,#6497,.T.);
#13705=EDGE_CURVE('',#10439,#10440,#579,.T.);
#13706=EDGE_CURVE('',#10440,#10435,#580,.T.);
#13707=EDGE_CURVE('',#10441,#10434,#581,.T.);
#13708=EDGE_CURVE('',#10438,#10441,#582,.T.);
#13709=EDGE_CURVE('',#10442,#10443,#6498,.T.);
#13710=EDGE_CURVE('',#10443,#10444,#583,.T.);
#13711=EDGE_CURVE('',#10444,#10439,#584,.T.);
#13712=EDGE_CURVE('',#10445,#10438,#585,.T.);
#13713=EDGE_CURVE('',#10442,#10445,#586,.T.);
#13714=EDGE_CURVE('',#10446,#10447,#6499,.T.);
#13715=EDGE_CURVE('',#10447,#10448,#587,.T.);
#13716=EDGE_CURVE('',#10448,#10443,#588,.T.);
#13717=EDGE_CURVE('',#10449,#10442,#589,.T.);
#13718=EDGE_CURVE('',#10446,#10449,#590,.T.);
#13719=EDGE_CURVE('',#10450,#10451,#6500,.T.);
#13720=EDGE_CURVE('',#10451,#10452,#591,.T.);
#13721=EDGE_CURVE('',#10452,#10447,#592,.T.);
#13722=EDGE_CURVE('',#10453,#10446,#593,.T.);
#13723=EDGE_CURVE('',#10450,#10453,#594,.T.);
#13724=EDGE_CURVE('',#10454,#10455,#6501,.T.);
#13725=EDGE_CURVE('',#10456,#10454,#595,.T.);
#13726=EDGE_CURVE('',#10457,#10456,#596,.T.);
#13727=EDGE_CURVE('',#10458,#10457,#5709,.T.);
#13728=EDGE_CURVE('',#10458,#10459,#597,.T.);
#13729=EDGE_CURVE('',#10459,#10455,#598,.T.);
#13730=EDGE_CURVE('',#10460,#10461,#6502,.T.);
#13731=EDGE_CURVE('',#10461,#10462,#599,.T.);
#13732=EDGE_CURVE('',#10462,#10463,#600,.T.);
#13733=EDGE_CURVE('',#10464,#10463,#5710,.T.);
#13734=EDGE_CURVE('',#10465,#10464,#601,.T.);
#13735=EDGE_CURVE('',#10460,#10465,#602,.T.);
#13736=EDGE_CURVE('',#10466,#10467,#6503,.T.);
#13737=EDGE_CURVE('',#10467,#10468,#603,.T.);
#13738=EDGE_CURVE('',#10468,#10461,#604,.T.);
#13739=EDGE_CURVE('',#10469,#10460,#605,.T.);
#13740=EDGE_CURVE('',#10466,#10469,#606,.T.);
#13741=EDGE_CURVE('',#10470,#10471,#6504,.T.);
#13742=EDGE_CURVE('',#10471,#10472,#607,.T.);
#13743=EDGE_CURVE('',#10472,#10467,#608,.T.);
#13744=EDGE_CURVE('',#10473,#10466,#609,.T.);
#13745=EDGE_CURVE('',#10470,#10473,#610,.T.);
#13746=EDGE_CURVE('',#10474,#10475,#6505,.T.);
#13747=EDGE_CURVE('',#10475,#10476,#611,.T.);
#13748=EDGE_CURVE('',#10476,#10471,#612,.T.);
#13749=EDGE_CURVE('',#10477,#10470,#613,.T.);
#13750=EDGE_CURVE('',#10474,#10477,#614,.T.);
#13751=EDGE_CURVE('',#10478,#10479,#6506,.T.);
#13752=EDGE_CURVE('',#10479,#10480,#615,.T.);
#13753=EDGE_CURVE('',#10480,#10475,#616,.T.);
#13754=EDGE_CURVE('',#10481,#10474,#617,.T.);
#13755=EDGE_CURVE('',#10478,#10481,#618,.T.);
#13756=EDGE_CURVE('',#10482,#10483,#6507,.T.);
#13757=EDGE_CURVE('',#10483,#10484,#619,.T.);
#13758=EDGE_CURVE('',#10484,#10479,#620,.T.);
#13759=EDGE_CURVE('',#10485,#10478,#621,.T.);
#13760=EDGE_CURVE('',#10482,#10485,#622,.T.);
#13761=EDGE_CURVE('',#10486,#10487,#6508,.T.);
#13762=EDGE_CURVE('',#10487,#10488,#623,.T.);
#13763=EDGE_CURVE('',#10488,#10483,#624,.T.);
#13764=EDGE_CURVE('',#10489,#10482,#625,.T.);
#13765=EDGE_CURVE('',#10486,#10489,#626,.T.);
#13766=EDGE_CURVE('',#10490,#10491,#6509,.T.);
#13767=EDGE_CURVE('',#10491,#10492,#627,.T.);
#13768=EDGE_CURVE('',#10492,#10487,#628,.T.);
#13769=EDGE_CURVE('',#10493,#10486,#629,.T.);
#13770=EDGE_CURVE('',#10490,#10493,#630,.T.);
#13771=EDGE_CURVE('',#10494,#10495,#6510,.T.);
#13772=EDGE_CURVE('',#10495,#10496,#631,.T.);
#13773=EDGE_CURVE('',#10496,#10491,#632,.T.);
#13774=EDGE_CURVE('',#10497,#10490,#633,.T.);
#13775=EDGE_CURVE('',#10494,#10497,#634,.T.);
#13776=EDGE_CURVE('',#10498,#10499,#6511,.T.);
#13777=EDGE_CURVE('',#10499,#10500,#635,.T.);
#13778=EDGE_CURVE('',#10500,#10495,#636,.T.);
#13779=EDGE_CURVE('',#10501,#10494,#637,.T.);
#13780=EDGE_CURVE('',#10498,#10501,#638,.T.);
#13781=EDGE_CURVE('',#10502,#10503,#6512,.T.);
#13782=EDGE_CURVE('',#10503,#10504,#639,.T.);
#13783=EDGE_CURVE('',#10504,#10499,#640,.T.);
#13784=EDGE_CURVE('',#10505,#10498,#641,.T.);
#13785=EDGE_CURVE('',#10502,#10505,#642,.T.);
#13786=EDGE_CURVE('',#10506,#10507,#6513,.T.);
#13787=EDGE_CURVE('',#10507,#10508,#643,.T.);
#13788=EDGE_CURVE('',#10508,#10503,#644,.T.);
#13789=EDGE_CURVE('',#10509,#10502,#645,.T.);
#13790=EDGE_CURVE('',#10506,#10509,#646,.T.);
#13791=EDGE_CURVE('',#10510,#10511,#6514,.T.);
#13792=EDGE_CURVE('',#10511,#10512,#647,.T.);
#13793=EDGE_CURVE('',#10512,#10507,#648,.T.);
#13794=EDGE_CURVE('',#10513,#10506,#649,.T.);
#13795=EDGE_CURVE('',#10510,#10513,#650,.T.);
#13796=EDGE_CURVE('',#10514,#10515,#6515,.T.);
#13797=EDGE_CURVE('',#10515,#10516,#651,.T.);
#13798=EDGE_CURVE('',#10516,#10511,#652,.T.);
#13799=EDGE_CURVE('',#10517,#10510,#653,.T.);
#13800=EDGE_CURVE('',#10514,#10517,#654,.T.);
#13801=EDGE_CURVE('',#10518,#10519,#6516,.T.);
#13802=EDGE_CURVE('',#10519,#10520,#655,.T.);
#13803=EDGE_CURVE('',#10520,#10515,#656,.T.);
#13804=EDGE_CURVE('',#10521,#10514,#657,.T.);
#13805=EDGE_CURVE('',#10518,#10521,#658,.T.);
#13806=EDGE_CURVE('',#10522,#10523,#6517,.T.);
#13807=EDGE_CURVE('',#10523,#10524,#659,.T.);
#13808=EDGE_CURVE('',#10524,#10519,#660,.T.);
#13809=EDGE_CURVE('',#10525,#10518,#661,.T.);
#13810=EDGE_CURVE('',#10522,#10525,#662,.T.);
#13811=EDGE_CURVE('',#10526,#10527,#6518,.T.);
#13812=EDGE_CURVE('',#10527,#10528,#663,.T.);
#13813=EDGE_CURVE('',#10528,#10523,#664,.T.);
#13814=EDGE_CURVE('',#10529,#10522,#665,.T.);
#13815=EDGE_CURVE('',#10526,#10529,#666,.T.);
#13816=EDGE_CURVE('',#10530,#10531,#6519,.T.);
#13817=EDGE_CURVE('',#10531,#10532,#667,.T.);
#13818=EDGE_CURVE('',#10532,#10527,#668,.T.);
#13819=EDGE_CURVE('',#10533,#10526,#669,.T.);
#13820=EDGE_CURVE('',#10530,#10533,#670,.T.);
#13821=EDGE_CURVE('',#10534,#10535,#6520,.T.);
#13822=EDGE_CURVE('',#10535,#10536,#671,.T.);
#13823=EDGE_CURVE('',#10536,#10531,#672,.T.);
#13824=EDGE_CURVE('',#10537,#10530,#673,.T.);
#13825=EDGE_CURVE('',#10534,#10537,#674,.T.);
#13826=EDGE_CURVE('',#10538,#10539,#6521,.T.);
#13827=EDGE_CURVE('',#10539,#10540,#675,.T.);
#13828=EDGE_CURVE('',#10540,#10535,#676,.T.);
#13829=EDGE_CURVE('',#10541,#10534,#677,.T.);
#13830=EDGE_CURVE('',#10538,#10541,#678,.T.);
#13831=EDGE_CURVE('',#10542,#10543,#6522,.T.);
#13832=EDGE_CURVE('',#10543,#10544,#679,.T.);
#13833=EDGE_CURVE('',#10544,#10539,#680,.T.);
#13834=EDGE_CURVE('',#10545,#10538,#681,.T.);
#13835=EDGE_CURVE('',#10542,#10545,#682,.T.);
#13836=EDGE_CURVE('',#10546,#10547,#6523,.T.);
#13837=EDGE_CURVE('',#10547,#10548,#683,.T.);
#13838=EDGE_CURVE('',#10548,#10543,#684,.T.);
#13839=EDGE_CURVE('',#10549,#10542,#685,.T.);
#13840=EDGE_CURVE('',#10546,#10549,#686,.T.);
#13841=EDGE_CURVE('',#10550,#10551,#6524,.T.);
#13842=EDGE_CURVE('',#10551,#10552,#687,.T.);
#13843=EDGE_CURVE('',#10552,#10547,#688,.T.);
#13844=EDGE_CURVE('',#10553,#10546,#689,.T.);
#13845=EDGE_CURVE('',#10550,#10553,#690,.T.);
#13846=EDGE_CURVE('',#10554,#10555,#6525,.T.);
#13847=EDGE_CURVE('',#10555,#10556,#691,.T.);
#13848=EDGE_CURVE('',#10556,#10551,#692,.T.);
#13849=EDGE_CURVE('',#10557,#10550,#693,.T.);
#13850=EDGE_CURVE('',#10554,#10557,#694,.T.);
#13851=EDGE_CURVE('',#10558,#10559,#6526,.T.);
#13852=EDGE_CURVE('',#10559,#10560,#695,.T.);
#13853=EDGE_CURVE('',#10560,#10555,#696,.T.);
#13854=EDGE_CURVE('',#10561,#10554,#697,.T.);
#13855=EDGE_CURVE('',#10558,#10561,#698,.T.);
#13856=EDGE_CURVE('',#10562,#10563,#6527,.T.);
#13857=EDGE_CURVE('',#10563,#10564,#699,.T.);
#13858=EDGE_CURVE('',#10564,#10559,#700,.T.);
#13859=EDGE_CURVE('',#10565,#10558,#701,.T.);
#13860=EDGE_CURVE('',#10562,#10565,#702,.T.);
#13861=EDGE_CURVE('',#10566,#10567,#6528,.T.);
#13862=EDGE_CURVE('',#10568,#10566,#703,.T.);
#13863=EDGE_CURVE('',#10569,#10568,#704,.T.);
#13864=EDGE_CURVE('',#10570,#10569,#5711,.T.);
#13865=EDGE_CURVE('',#10570,#10571,#705,.T.);
#13866=EDGE_CURVE('',#10571,#10567,#706,.T.);
#13867=EDGE_CURVE('',#10572,#10573,#6529,.T.);
#13868=EDGE_CURVE('',#10573,#10574,#707,.F.);
#13869=EDGE_CURVE('',#10574,#10575,#5712,.F.);
#13870=EDGE_CURVE('',#10575,#10576,#708,.T.);
#13871=EDGE_CURVE('',#10576,#10572,#709,.T.);
#13872=EDGE_CURVE('',#10577,#10578,#6530,.T.);
#13873=EDGE_CURVE('',#10578,#10579,#710,.T.);
#13874=EDGE_CURVE('',#10579,#10573,#711,.F.);
#13875=EDGE_CURVE('',#10572,#10580,#712,.T.);
#13876=EDGE_CURVE('',#10580,#10577,#713,.T.);
#13877=EDGE_CURVE('',#10581,#10582,#6531,.T.);
#13878=EDGE_CURVE('',#10582,#10583,#714,.T.);
#13879=EDGE_CURVE('',#10583,#10578,#715,.T.);
#13880=EDGE_CURVE('',#10577,#10584,#716,.T.);
#13881=EDGE_CURVE('',#10584,#10581,#717,.T.);
#13882=EDGE_CURVE('',#10585,#10586,#6532,.T.);
#13883=EDGE_CURVE('',#10587,#10585,#5713,.F.);
#13884=EDGE_CURVE('',#10587,#10586,#718,.T.);
#13885=EDGE_CURVE('',#10588,#10589,#6533,.T.);
#13886=EDGE_CURVE('',#10589,#10590,#5714,.T.);
#13887=EDGE_CURVE('',#10590,#10588,#719,.T.);
#13888=EDGE_CURVE('',#10591,#10592,#6534,.T.);
#13889=EDGE_CURVE('',#10592,#10593,#720,.T.);
#13890=EDGE_CURVE('',#10593,#10589,#5715,.T.);
#13891=EDGE_CURVE('',#10588,#10591,#721,.T.);
#13892=EDGE_CURVE('',#10594,#10595,#6535,.T.);
#13893=EDGE_CURVE('',#10595,#10596,#722,.T.);
#13894=EDGE_CURVE('',#10596,#10592,#723,.T.);
#13895=EDGE_CURVE('',#10591,#10597,#724,.T.);
#13896=EDGE_CURVE('',#10597,#10594,#725,.T.);
#13897=EDGE_CURVE('',#10598,#10599,#6536,.T.);
#13898=EDGE_CURVE('',#10598,#10600,#726,.F.);
#13899=EDGE_CURVE('',#10600,#10601,#5716,.F.);
#13900=EDGE_CURVE('',#10601,#10602,#727,.T.);
#13901=EDGE_CURVE('',#10602,#10599,#728,.T.);
#13902=EDGE_CURVE('',#10603,#10604,#6537,.T.);
#13903=EDGE_CURVE('',#10604,#10605,#729,.T.);
#13904=EDGE_CURVE('',#10605,#10606,#730,.T.);
#13905=EDGE_CURVE('',#10607,#10606,#5717,.T.);
#13906=EDGE_CURVE('',#10607,#10608,#731,.T.);
#13907=EDGE_CURVE('',#10608,#10603,#732,.T.);
#13908=EDGE_CURVE('',#10609,#10610,#6538,.T.);
#13909=EDGE_CURVE('',#10610,#10604,#733,.T.);
#13910=EDGE_CURVE('',#10603,#10609,#734,.T.);
#13911=EDGE_CURVE('',#10611,#10612,#6539,.T.);
#13912=EDGE_CURVE('',#10612,#10613,#735,.T.);
#13913=EDGE_CURVE('',#10613,#10610,#736,.T.);
#13914=EDGE_CURVE('',#10609,#10614,#737,.T.);
#13915=EDGE_CURVE('',#10614,#10611,#738,.T.);
#13916=EDGE_CURVE('',#10615,#10616,#6540,.T.);
#13917=EDGE_CURVE('',#10616,#10617,#739,.T.);
#13918=EDGE_CURVE('',#10617,#10612,#740,.T.);
#13919=EDGE_CURVE('',#10611,#10615,#741,.T.);
#13920=EDGE_CURVE('',#10618,#10619,#6541,.T.);
#13921=EDGE_CURVE('',#10619,#10620,#742,.T.);
#13922=EDGE_CURVE('',#10620,#10616,#743,.T.);
#13923=EDGE_CURVE('',#10615,#10621,#744,.T.);
#13924=EDGE_CURVE('',#10621,#10618,#745,.T.);
#13925=EDGE_CURVE('',#10622,#10623,#6542,.T.);
#13926=EDGE_CURVE('',#10623,#10619,#746,.T.);
#13927=EDGE_CURVE('',#10618,#10622,#747,.T.);
#13928=EDGE_CURVE('',#10624,#10625,#6543,.T.);
#13929=EDGE_CURVE('',#10625,#10626,#748,.T.);
#13930=EDGE_CURVE('',#10626,#10623,#749,.T.);
#13931=EDGE_CURVE('',#10622,#10627,#750,.T.);
#13932=EDGE_CURVE('',#10627,#10624,#751,.T.);
#13933=EDGE_CURVE('',#10628,#10629,#6544,.T.);
#13934=EDGE_CURVE('',#10629,#10625,#752,.T.);
#13935=EDGE_CURVE('',#10624,#10628,#753,.T.);
#13936=EDGE_CURVE('',#10630,#10631,#6545,.T.);
#13937=EDGE_CURVE('',#10631,#10632,#754,.T.);
#13938=EDGE_CURVE('',#10632,#10629,#755,.T.);
#13939=EDGE_CURVE('',#10628,#10633,#756,.T.);
#13940=EDGE_CURVE('',#10633,#10630,#757,.T.);
#13941=EDGE_CURVE('',#10634,#10635,#6546,.T.);
#13942=EDGE_CURVE('',#10635,#10636,#758,.T.);
#13943=EDGE_CURVE('',#10636,#10631,#759,.T.);
#13944=EDGE_CURVE('',#10630,#10634,#760,.T.);
#13945=EDGE_CURVE('',#10637,#10638,#6547,.T.);
#13946=EDGE_CURVE('',#10638,#10639,#761,.T.);
#13947=EDGE_CURVE('',#10639,#10635,#762,.T.);
#13948=EDGE_CURVE('',#10634,#10640,#763,.T.);
#13949=EDGE_CURVE('',#10640,#10637,#764,.T.);
#13950=EDGE_CURVE('',#10641,#10642,#6548,.T.);
#13951=EDGE_CURVE('',#10642,#10638,#765,.T.);
#13952=EDGE_CURVE('',#10637,#10643,#766,.T.);
#13953=EDGE_CURVE('',#10643,#10641,#767,.T.);
#13954=EDGE_CURVE('',#10644,#10645,#6549,.T.);
#13955=EDGE_CURVE('',#10645,#10646,#768,.T.);
#13956=EDGE_CURVE('',#10646,#10642,#769,.T.);
#13957=EDGE_CURVE('',#10641,#10647,#770,.T.);
#13958=EDGE_CURVE('',#10647,#10644,#771,.T.);
#13959=EDGE_CURVE('',#10648,#10649,#6550,.T.);
#13960=EDGE_CURVE('',#10649,#10645,#772,.T.);
#13961=EDGE_CURVE('',#10644,#10648,#773,.T.);
#13962=EDGE_CURVE('',#10650,#10651,#6551,.T.);
#13963=EDGE_CURVE('',#10651,#10652,#774,.T.);
#13964=EDGE_CURVE('',#10652,#10649,#775,.T.);
#13965=EDGE_CURVE('',#10648,#10653,#776,.T.);
#13966=EDGE_CURVE('',#10653,#10650,#777,.T.);
#13967=EDGE_CURVE('',#10654,#10655,#6552,.T.);
#13968=EDGE_CURVE('',#10655,#10656,#778,.T.);
#13969=EDGE_CURVE('',#10656,#10651,#779,.T.);
#13970=EDGE_CURVE('',#10650,#10654,#780,.T.);
#13971=EDGE_CURVE('',#10657,#10658,#6553,.T.);
#13972=EDGE_CURVE('',#10658,#10659,#781,.T.);
#13973=EDGE_CURVE('',#10659,#10655,#782,.T.);
#13974=EDGE_CURVE('',#10654,#10660,#783,.T.);
#13975=EDGE_CURVE('',#10660,#10657,#784,.T.);
#13976=EDGE_CURVE('',#10661,#10662,#6554,.T.);
#13977=EDGE_CURVE('',#10662,#10658,#785,.T.);
#13978=EDGE_CURVE('',#10657,#10663,#786,.T.);
#13979=EDGE_CURVE('',#10663,#10661,#787,.T.);
#13980=EDGE_CURVE('',#10664,#10665,#6555,.T.);
#13981=EDGE_CURVE('',#10665,#10666,#788,.T.);
#13982=EDGE_CURVE('',#10666,#10662,#789,.T.);
#13983=EDGE_CURVE('',#10661,#10667,#790,.T.);
#13984=EDGE_CURVE('',#10667,#10664,#791,.T.);
#13985=EDGE_CURVE('',#10668,#10669,#6556,.T.);
#13986=EDGE_CURVE('',#10669,#10665,#792,.T.);
#13987=EDGE_CURVE('',#10664,#10668,#793,.T.);
#13988=EDGE_CURVE('',#10670,#10671,#6557,.T.);
#13989=EDGE_CURVE('',#10671,#10672,#794,.T.);
#13990=EDGE_CURVE('',#10672,#10669,#795,.T.);
#13991=EDGE_CURVE('',#10668,#10673,#796,.T.);
#13992=EDGE_CURVE('',#10673,#10670,#797,.T.);
#13993=EDGE_CURVE('',#10674,#10675,#6558,.T.);
#13994=EDGE_CURVE('',#10675,#10671,#798,.T.);
#13995=EDGE_CURVE('',#10670,#10674,#799,.T.);
#13996=EDGE_CURVE('',#10676,#10677,#6559,.T.);
#13997=EDGE_CURVE('',#10677,#10678,#800,.T.);
#13998=EDGE_CURVE('',#10678,#10675,#801,.T.);
#13999=EDGE_CURVE('',#10674,#10679,#802,.T.);
#14000=EDGE_CURVE('',#10679,#10676,#803,.T.);
#14001=EDGE_CURVE('',#10680,#10681,#6560,.T.);
#14002=EDGE_CURVE('',#10681,#10677,#804,.T.);
#14003=EDGE_CURVE('',#10676,#10682,#805,.T.);
#14004=EDGE_CURVE('',#10682,#10680,#806,.T.);
#14005=EDGE_CURVE('',#10683,#10684,#6561,.T.);
#14006=EDGE_CURVE('',#10684,#10685,#807,.T.);
#14007=EDGE_CURVE('',#10685,#10681,#808,.T.);
#14008=EDGE_CURVE('',#10680,#10686,#809,.T.);
#14009=EDGE_CURVE('',#10686,#10683,#810,.T.);
#14010=EDGE_CURVE('',#10687,#10688,#6562,.T.);
#14011=EDGE_CURVE('',#10688,#10684,#811,.T.);
#14012=EDGE_CURVE('',#10683,#10687,#812,.T.);
#14013=EDGE_CURVE('',#10689,#10690,#6563,.T.);
#14014=EDGE_CURVE('',#10689,#10691,#813,.T.);
#14015=EDGE_CURVE('',#10692,#10691,#5718,.F.);
#14016=EDGE_CURVE('',#10692,#10690,#814,.T.);
#14017=EDGE_CURVE('',#10693,#10694,#6564,.T.);
#14018=EDGE_CURVE('',#10694,#10695,#815,.T.);
#14019=EDGE_CURVE('',#10695,#10696,#816,.T.);
#14020=EDGE_CURVE('',#10697,#10696,#5719,.T.);
#14021=EDGE_CURVE('',#10697,#10698,#817,.T.);
#14022=EDGE_CURVE('',#10698,#10693,#818,.T.);
#14023=EDGE_CURVE('',#10699,#10700,#6565,.T.);
#14024=EDGE_CURVE('',#10700,#10694,#819,.T.);
#14025=EDGE_CURVE('',#10693,#10699,#820,.T.);
#14026=EDGE_CURVE('',#10701,#10702,#6566,.T.);
#14027=EDGE_CURVE('',#10702,#10703,#821,.T.);
#14028=EDGE_CURVE('',#10703,#10700,#822,.T.);
#14029=EDGE_CURVE('',#10699,#10704,#823,.T.);
#14030=EDGE_CURVE('',#10704,#10701,#824,.T.);
#14031=EDGE_CURVE('',#10705,#10706,#6567,.T.);
#14032=EDGE_CURVE('',#10706,#10707,#825,.T.);
#14033=EDGE_CURVE('',#10707,#10702,#826,.T.);
#14034=EDGE_CURVE('',#10701,#10705,#827,.T.);
#14035=EDGE_CURVE('',#10708,#10709,#6568,.T.);
#14036=EDGE_CURVE('',#10709,#10710,#828,.T.);
#14037=EDGE_CURVE('',#10710,#10706,#829,.T.);
#14038=EDGE_CURVE('',#10705,#10711,#830,.T.);
#14039=EDGE_CURVE('',#10711,#10708,#831,.T.);
#14040=EDGE_CURVE('',#10712,#10713,#6569,.T.);
#14041=EDGE_CURVE('',#10713,#10709,#832,.T.);
#14042=EDGE_CURVE('',#10708,#10712,#833,.T.);
#14043=EDGE_CURVE('',#10714,#10715,#6570,.T.);
#14044=EDGE_CURVE('',#10715,#10716,#834,.T.);
#14045=EDGE_CURVE('',#10716,#10713,#835,.T.);
#14046=EDGE_CURVE('',#10712,#10717,#836,.T.);
#14047=EDGE_CURVE('',#10717,#10714,#837,.T.);
#14048=EDGE_CURVE('',#10718,#10719,#6571,.T.);
#14049=EDGE_CURVE('',#10719,#10715,#838,.T.);
#14050=EDGE_CURVE('',#10714,#10718,#839,.T.);
#14051=EDGE_CURVE('',#10720,#10721,#6572,.T.);
#14052=EDGE_CURVE('',#10721,#10722,#840,.T.);
#14053=EDGE_CURVE('',#10722,#10719,#841,.T.);
#14054=EDGE_CURVE('',#10718,#10723,#842,.T.);
#14055=EDGE_CURVE('',#10723,#10720,#843,.T.);
#14056=EDGE_CURVE('',#10724,#10725,#6573,.T.);
#14057=EDGE_CURVE('',#10725,#10726,#844,.T.);
#14058=EDGE_CURVE('',#10726,#10721,#845,.T.);
#14059=EDGE_CURVE('',#10720,#10724,#846,.T.);
#14060=EDGE_CURVE('',#10727,#10728,#6574,.T.);
#14061=EDGE_CURVE('',#10728,#10729,#847,.T.);
#14062=EDGE_CURVE('',#10729,#10725,#848,.T.);
#14063=EDGE_CURVE('',#10724,#10730,#849,.T.);
#14064=EDGE_CURVE('',#10730,#10727,#850,.T.);
#14065=EDGE_CURVE('',#10731,#10732,#6575,.T.);
#14066=EDGE_CURVE('',#10732,#10728,#851,.T.);
#14067=EDGE_CURVE('',#10727,#10733,#852,.T.);
#14068=EDGE_CURVE('',#10733,#10731,#853,.T.);
#14069=EDGE_CURVE('',#10734,#10735,#6576,.T.);
#14070=EDGE_CURVE('',#10735,#10736,#854,.T.);
#14071=EDGE_CURVE('',#10736,#10732,#855,.T.);
#14072=EDGE_CURVE('',#10731,#10737,#856,.T.);
#14073=EDGE_CURVE('',#10737,#10734,#857,.T.);
#14074=EDGE_CURVE('',#10738,#10739,#6577,.T.);
#14075=EDGE_CURVE('',#10739,#10735,#858,.T.);
#14076=EDGE_CURVE('',#10734,#10738,#859,.T.);
#14077=EDGE_CURVE('',#10740,#10741,#6578,.T.);
#14078=EDGE_CURVE('',#10741,#10742,#860,.T.);
#14079=EDGE_CURVE('',#10742,#10739,#861,.T.);
#14080=EDGE_CURVE('',#10738,#10743,#862,.T.);
#14081=EDGE_CURVE('',#10743,#10740,#863,.T.);
#14082=EDGE_CURVE('',#10744,#10745,#6579,.T.);
#14083=EDGE_CURVE('',#10745,#10746,#864,.T.);
#14084=EDGE_CURVE('',#10746,#10741,#865,.T.);
#14085=EDGE_CURVE('',#10740,#10744,#866,.T.);
#14086=EDGE_CURVE('',#10747,#10748,#6580,.T.);
#14087=EDGE_CURVE('',#10748,#10749,#867,.T.);
#14088=EDGE_CURVE('',#10749,#10745,#868,.T.);
#14089=EDGE_CURVE('',#10744,#10750,#869,.T.);
#14090=EDGE_CURVE('',#10750,#10747,#870,.T.);
#14091=EDGE_CURVE('',#10751,#10752,#6581,.T.);
#14092=EDGE_CURVE('',#10752,#10748,#871,.T.);
#14093=EDGE_CURVE('',#10747,#10753,#872,.T.);
#14094=EDGE_CURVE('',#10753,#10751,#873,.T.);
#14095=EDGE_CURVE('',#10754,#10755,#6582,.T.);
#14096=EDGE_CURVE('',#10755,#10756,#874,.T.);
#14097=EDGE_CURVE('',#10756,#10752,#875,.T.);
#14098=EDGE_CURVE('',#10751,#10757,#876,.T.);
#14099=EDGE_CURVE('',#10757,#10754,#877,.T.);
#14100=EDGE_CURVE('',#10758,#10759,#6583,.T.);
#14101=EDGE_CURVE('',#10759,#10755,#878,.T.);
#14102=EDGE_CURVE('',#10754,#10758,#879,.T.);
#14103=EDGE_CURVE('',#10760,#10761,#6584,.T.);
#14104=EDGE_CURVE('',#10761,#10762,#880,.T.);
#14105=EDGE_CURVE('',#10762,#10759,#881,.T.);
#14106=EDGE_CURVE('',#10758,#10763,#882,.T.);
#14107=EDGE_CURVE('',#10763,#10760,#883,.T.);
#14108=EDGE_CURVE('',#10764,#10765,#6585,.T.);
#14109=EDGE_CURVE('',#10765,#10761,#884,.T.);
#14110=EDGE_CURVE('',#10760,#10764,#885,.T.);
#14111=EDGE_CURVE('',#10766,#10767,#6586,.T.);
#14112=EDGE_CURVE('',#10767,#10768,#886,.T.);
#14113=EDGE_CURVE('',#10768,#10765,#887,.T.);
#14114=EDGE_CURVE('',#10764,#10769,#888,.T.);
#14115=EDGE_CURVE('',#10769,#10766,#889,.T.);
#14116=EDGE_CURVE('',#10770,#10771,#6587,.T.);
#14117=EDGE_CURVE('',#10771,#10767,#890,.T.);
#14118=EDGE_CURVE('',#10766,#10772,#891,.T.);
#14119=EDGE_CURVE('',#10772,#10770,#892,.T.);
#14120=EDGE_CURVE('',#10773,#10774,#6588,.T.);
#14121=EDGE_CURVE('',#10774,#10775,#893,.T.);
#14122=EDGE_CURVE('',#10775,#10771,#894,.T.);
#14123=EDGE_CURVE('',#10770,#10776,#895,.T.);
#14124=EDGE_CURVE('',#10776,#10773,#896,.T.);
#14125=EDGE_CURVE('',#10777,#10778,#6589,.T.);
#14126=EDGE_CURVE('',#10778,#10774,#897,.T.);
#14127=EDGE_CURVE('',#10773,#10777,#898,.T.);
#14128=EDGE_CURVE('',#10779,#10780,#6590,.T.);
#14129=EDGE_CURVE('',#10779,#10781,#899,.T.);
#14130=EDGE_CURVE('',#10782,#10781,#5720,.F.);
#14131=EDGE_CURVE('',#10782,#10780,#900,.T.);
#14132=EDGE_CURVE('',#10783,#10784,#6591,.T.);
#14133=EDGE_CURVE('',#10784,#10785,#901,.T.);
#14134=EDGE_CURVE('',#10785,#10786,#902,.T.);
#14135=EDGE_CURVE('',#10787,#10786,#5721,.T.);
#14136=EDGE_CURVE('',#10787,#10788,#903,.T.);
#14137=EDGE_CURVE('',#10788,#10783,#904,.T.);
#14138=EDGE_CURVE('',#10789,#10790,#6592,.T.);
#14139=EDGE_CURVE('',#10790,#10784,#905,.T.);
#14140=EDGE_CURVE('',#10783,#10789,#906,.T.);
#14141=EDGE_CURVE('',#10791,#10792,#6593,.T.);
#14142=EDGE_CURVE('',#10792,#10793,#907,.T.);
#14143=EDGE_CURVE('',#10793,#10790,#908,.T.);
#14144=EDGE_CURVE('',#10789,#10794,#909,.T.);
#14145=EDGE_CURVE('',#10794,#10791,#910,.T.);
#14146=EDGE_CURVE('',#10795,#10796,#6594,.T.);
#14147=EDGE_CURVE('',#10796,#10797,#911,.T.);
#14148=EDGE_CURVE('',#10797,#10792,#912,.T.);
#14149=EDGE_CURVE('',#10791,#10795,#913,.T.);
#14150=EDGE_CURVE('',#10798,#10799,#6595,.T.);
#14151=EDGE_CURVE('',#10799,#10800,#914,.T.);
#14152=EDGE_CURVE('',#10800,#10796,#915,.T.);
#14153=EDGE_CURVE('',#10795,#10801,#916,.T.);
#14154=EDGE_CURVE('',#10801,#10798,#917,.T.);
#14155=EDGE_CURVE('',#10802,#10803,#6596,.T.);
#14156=EDGE_CURVE('',#10803,#10799,#918,.T.);
#14157=EDGE_CURVE('',#10798,#10802,#919,.T.);
#14158=EDGE_CURVE('',#10804,#10805,#6597,.T.);
#14159=EDGE_CURVE('',#10805,#10806,#920,.T.);
#14160=EDGE_CURVE('',#10806,#10803,#921,.T.);
#14161=EDGE_CURVE('',#10802,#10807,#922,.T.);
#14162=EDGE_CURVE('',#10807,#10804,#923,.T.);
#14163=EDGE_CURVE('',#10808,#10809,#6598,.T.);
#14164=EDGE_CURVE('',#10809,#10805,#924,.T.);
#14165=EDGE_CURVE('',#10804,#10808,#925,.T.);
#14166=EDGE_CURVE('',#10810,#10811,#6599,.T.);
#14167=EDGE_CURVE('',#10811,#10812,#926,.T.);
#14168=EDGE_CURVE('',#10812,#10809,#927,.T.);
#14169=EDGE_CURVE('',#10808,#10813,#928,.T.);
#14170=EDGE_CURVE('',#10813,#10810,#929,.T.);
#14171=EDGE_CURVE('',#10814,#10815,#6600,.T.);
#14172=EDGE_CURVE('',#10815,#10816,#930,.T.);
#14173=EDGE_CURVE('',#10816,#10811,#931,.T.);
#14174=EDGE_CURVE('',#10810,#10814,#932,.T.);
#14175=EDGE_CURVE('',#10817,#10818,#6601,.T.);
#14176=EDGE_CURVE('',#10818,#10819,#933,.T.);
#14177=EDGE_CURVE('',#10819,#10815,#934,.T.);
#14178=EDGE_CURVE('',#10814,#10820,#935,.T.);
#14179=EDGE_CURVE('',#10820,#10817,#936,.T.);
#14180=EDGE_CURVE('',#10821,#10822,#6602,.T.);
#14181=EDGE_CURVE('',#10822,#10818,#937,.T.);
#14182=EDGE_CURVE('',#10817,#10823,#938,.T.);
#14183=EDGE_CURVE('',#10823,#10821,#939,.T.);
#14184=EDGE_CURVE('',#10824,#10825,#6603,.T.);
#14185=EDGE_CURVE('',#10825,#10826,#940,.T.);
#14186=EDGE_CURVE('',#10826,#10822,#941,.T.);
#14187=EDGE_CURVE('',#10821,#10827,#942,.T.);
#14188=EDGE_CURVE('',#10827,#10824,#943,.T.);
#14189=EDGE_CURVE('',#10828,#10829,#6604,.T.);
#14190=EDGE_CURVE('',#10829,#10825,#944,.T.);
#14191=EDGE_CURVE('',#10824,#10828,#945,.T.);
#14192=EDGE_CURVE('',#10830,#10831,#6605,.T.);
#14193=EDGE_CURVE('',#10831,#10832,#946,.T.);
#14194=EDGE_CURVE('',#10832,#10829,#947,.T.);
#14195=EDGE_CURVE('',#10828,#10833,#948,.T.);
#14196=EDGE_CURVE('',#10833,#10830,#949,.T.);
#14197=EDGE_CURVE('',#10834,#10835,#6606,.T.);
#14198=EDGE_CURVE('',#10835,#10836,#950,.T.);
#14199=EDGE_CURVE('',#10836,#10831,#951,.T.);
#14200=EDGE_CURVE('',#10830,#10834,#952,.T.);
#14201=EDGE_CURVE('',#10837,#10838,#6607,.T.);
#14202=EDGE_CURVE('',#10838,#10839,#953,.T.);
#14203=EDGE_CURVE('',#10839,#10835,#954,.T.);
#14204=EDGE_CURVE('',#10834,#10840,#955,.T.);
#14205=EDGE_CURVE('',#10840,#10837,#956,.T.);
#14206=EDGE_CURVE('',#10841,#10842,#6608,.T.);
#14207=EDGE_CURVE('',#10842,#10838,#957,.T.);
#14208=EDGE_CURVE('',#10837,#10843,#958,.T.);
#14209=EDGE_CURVE('',#10843,#10841,#959,.T.);
#14210=EDGE_CURVE('',#10844,#10845,#6609,.T.);
#14211=EDGE_CURVE('',#10845,#10846,#960,.T.);
#14212=EDGE_CURVE('',#10846,#10842,#961,.T.);
#14213=EDGE_CURVE('',#10841,#10847,#962,.T.);
#14214=EDGE_CURVE('',#10847,#10844,#963,.T.);
#14215=EDGE_CURVE('',#10848,#10849,#6610,.T.);
#14216=EDGE_CURVE('',#10849,#10845,#964,.T.);
#14217=EDGE_CURVE('',#10844,#10848,#965,.T.);
#14218=EDGE_CURVE('',#10850,#10851,#6611,.T.);
#14219=EDGE_CURVE('',#10851,#10852,#966,.T.);
#14220=EDGE_CURVE('',#10852,#10849,#967,.T.);
#14221=EDGE_CURVE('',#10848,#10853,#968,.T.);
#14222=EDGE_CURVE('',#10853,#10850,#969,.T.);
#14223=EDGE_CURVE('',#10854,#10855,#6612,.T.);
#14224=EDGE_CURVE('',#10855,#10851,#970,.T.);
#14225=EDGE_CURVE('',#10850,#10854,#971,.T.);
#14226=EDGE_CURVE('',#10856,#10857,#6613,.T.);
#14227=EDGE_CURVE('',#10857,#10858,#972,.T.);
#14228=EDGE_CURVE('',#10858,#10855,#973,.T.);
#14229=EDGE_CURVE('',#10854,#10859,#974,.T.);
#14230=EDGE_CURVE('',#10859,#10856,#975,.T.);
#14231=EDGE_CURVE('',#10860,#10861,#6614,.T.);
#14232=EDGE_CURVE('',#10861,#10857,#976,.T.);
#14233=EDGE_CURVE('',#10856,#10862,#977,.T.);
#14234=EDGE_CURVE('',#10862,#10860,#978,.T.);
#14235=EDGE_CURVE('',#10863,#10864,#6615,.T.);
#14236=EDGE_CURVE('',#10864,#10865,#979,.T.);
#14237=EDGE_CURVE('',#10865,#10861,#980,.T.);
#14238=EDGE_CURVE('',#10860,#10866,#981,.T.);
#14239=EDGE_CURVE('',#10866,#10863,#982,.T.);
#14240=EDGE_CURVE('',#10867,#10868,#6616,.T.);
#14241=EDGE_CURVE('',#10868,#10864,#983,.T.);
#14242=EDGE_CURVE('',#10863,#10867,#984,.T.);
#14243=EDGE_CURVE('',#10869,#10870,#6617,.T.);
#14244=EDGE_CURVE('',#10869,#10871,#985,.T.);
#14245=EDGE_CURVE('',#10872,#10871,#5722,.F.);
#14246=EDGE_CURVE('',#10872,#10870,#986,.T.);
#14247=EDGE_CURVE('',#10873,#10874,#6618,.T.);
#14248=EDGE_CURVE('',#10874,#10875,#987,.T.);
#14249=EDGE_CURVE('',#10875,#10876,#988,.T.);
#14250=EDGE_CURVE('',#10877,#10876,#5723,.T.);
#14251=EDGE_CURVE('',#10877,#10878,#989,.T.);
#14252=EDGE_CURVE('',#10878,#10873,#990,.T.);
#14253=EDGE_CURVE('',#10879,#10880,#6619,.T.);
#14254=EDGE_CURVE('',#10880,#10874,#991,.T.);
#14255=EDGE_CURVE('',#10873,#10879,#992,.T.);
#14256=EDGE_CURVE('',#10881,#10882,#6620,.T.);
#14257=EDGE_CURVE('',#10882,#10883,#993,.T.);
#14258=EDGE_CURVE('',#10883,#10880,#994,.T.);
#14259=EDGE_CURVE('',#10879,#10884,#995,.T.);
#14260=EDGE_CURVE('',#10884,#10881,#996,.T.);
#14261=EDGE_CURVE('',#10885,#10886,#6621,.T.);
#14262=EDGE_CURVE('',#10886,#10887,#997,.T.);
#14263=EDGE_CURVE('',#10887,#10882,#998,.T.);
#14264=EDGE_CURVE('',#10881,#10885,#999,.T.);
#14265=EDGE_CURVE('',#10888,#10889,#6622,.T.);
#14266=EDGE_CURVE('',#10889,#10890,#1000,.T.);
#14267=EDGE_CURVE('',#10890,#10886,#1001,.T.);
#14268=EDGE_CURVE('',#10885,#10891,#1002,.T.);
#14269=EDGE_CURVE('',#10891,#10888,#1003,.T.);
#14270=EDGE_CURVE('',#10892,#10893,#6623,.T.);
#14271=EDGE_CURVE('',#10893,#10889,#1004,.T.);
#14272=EDGE_CURVE('',#10888,#10892,#1005,.T.);
#14273=EDGE_CURVE('',#10894,#10895,#6624,.T.);
#14274=EDGE_CURVE('',#10895,#10896,#1006,.T.);
#14275=EDGE_CURVE('',#10896,#10893,#1007,.T.);
#14276=EDGE_CURVE('',#10892,#10897,#1008,.T.);
#14277=EDGE_CURVE('',#10897,#10894,#1009,.T.);
#14278=EDGE_CURVE('',#10898,#10899,#6625,.T.);
#14279=EDGE_CURVE('',#10899,#10895,#1010,.T.);
#14280=EDGE_CURVE('',#10894,#10898,#1011,.T.);
#14281=EDGE_CURVE('',#10900,#10901,#6626,.T.);
#14282=EDGE_CURVE('',#10901,#10902,#1012,.T.);
#14283=EDGE_CURVE('',#10902,#10899,#1013,.T.);
#14284=EDGE_CURVE('',#10898,#10903,#1014,.T.);
#14285=EDGE_CURVE('',#10903,#10900,#1015,.T.);
#14286=EDGE_CURVE('',#10904,#10905,#6627,.T.);
#14287=EDGE_CURVE('',#10905,#10906,#1016,.T.);
#14288=EDGE_CURVE('',#10906,#10901,#1017,.T.);
#14289=EDGE_CURVE('',#10900,#10904,#1018,.T.);
#14290=EDGE_CURVE('',#10907,#10908,#6628,.T.);
#14291=EDGE_CURVE('',#10908,#10909,#1019,.T.);
#14292=EDGE_CURVE('',#10909,#10905,#1020,.T.);
#14293=EDGE_CURVE('',#10904,#10910,#1021,.T.);
#14294=EDGE_CURVE('',#10910,#10907,#1022,.T.);
#14295=EDGE_CURVE('',#10911,#10912,#6629,.T.);
#14296=EDGE_CURVE('',#10912,#10908,#1023,.T.);
#14297=EDGE_CURVE('',#10907,#10913,#1024,.T.);
#14298=EDGE_CURVE('',#10913,#10911,#1025,.T.);
#14299=EDGE_CURVE('',#10914,#10915,#6630,.T.);
#14300=EDGE_CURVE('',#10915,#10916,#1026,.T.);
#14301=EDGE_CURVE('',#10916,#10912,#1027,.T.);
#14302=EDGE_CURVE('',#10911,#10917,#1028,.T.);
#14303=EDGE_CURVE('',#10917,#10914,#1029,.T.);
#14304=EDGE_CURVE('',#10918,#10919,#6631,.T.);
#14305=EDGE_CURVE('',#10919,#10915,#1030,.T.);
#14306=EDGE_CURVE('',#10914,#10918,#1031,.T.);
#14307=EDGE_CURVE('',#10920,#10921,#6632,.T.);
#14308=EDGE_CURVE('',#10921,#10922,#1032,.T.);
#14309=EDGE_CURVE('',#10922,#10919,#1033,.T.);
#14310=EDGE_CURVE('',#10918,#10923,#1034,.T.);
#14311=EDGE_CURVE('',#10923,#10920,#1035,.T.);
#14312=EDGE_CURVE('',#10924,#10925,#6633,.T.);
#14313=EDGE_CURVE('',#10925,#10926,#1036,.T.);
#14314=EDGE_CURVE('',#10926,#10921,#1037,.T.);
#14315=EDGE_CURVE('',#10920,#10924,#1038,.T.);
#14316=EDGE_CURVE('',#10927,#10928,#6634,.T.);
#14317=EDGE_CURVE('',#10928,#10929,#1039,.T.);
#14318=EDGE_CURVE('',#10929,#10925,#1040,.T.);
#14319=EDGE_CURVE('',#10924,#10930,#1041,.T.);
#14320=EDGE_CURVE('',#10930,#10927,#1042,.T.);
#14321=EDGE_CURVE('',#10931,#10932,#6635,.T.);
#14322=EDGE_CURVE('',#10932,#10928,#1043,.T.);
#14323=EDGE_CURVE('',#10927,#10933,#1044,.T.);
#14324=EDGE_CURVE('',#10933,#10931,#1045,.T.);
#14325=EDGE_CURVE('',#10934,#10935,#6636,.T.);
#14326=EDGE_CURVE('',#10935,#10936,#1046,.T.);
#14327=EDGE_CURVE('',#10936,#10932,#1047,.T.);
#14328=EDGE_CURVE('',#10931,#10937,#1048,.T.);
#14329=EDGE_CURVE('',#10937,#10934,#1049,.T.);
#14330=EDGE_CURVE('',#10938,#10939,#6637,.T.);
#14331=EDGE_CURVE('',#10939,#10935,#1050,.T.);
#14332=EDGE_CURVE('',#10934,#10938,#1051,.T.);
#14333=EDGE_CURVE('',#10940,#10941,#6638,.T.);
#14334=EDGE_CURVE('',#10941,#10942,#1052,.T.);
#14335=EDGE_CURVE('',#10942,#10939,#1053,.T.);
#14336=EDGE_CURVE('',#10938,#10943,#1054,.T.);
#14337=EDGE_CURVE('',#10943,#10940,#1055,.T.);
#14338=EDGE_CURVE('',#10944,#10945,#6639,.T.);
#14339=EDGE_CURVE('',#10945,#10941,#1056,.T.);
#14340=EDGE_CURVE('',#10940,#10944,#1057,.T.);
#14341=EDGE_CURVE('',#10946,#10947,#6640,.T.);
#14342=EDGE_CURVE('',#10947,#10948,#1058,.T.);
#14343=EDGE_CURVE('',#10948,#10945,#1059,.T.);
#14344=EDGE_CURVE('',#10944,#10949,#1060,.T.);
#14345=EDGE_CURVE('',#10949,#10946,#1061,.T.);
#14346=EDGE_CURVE('',#10950,#10951,#6641,.T.);
#14347=EDGE_CURVE('',#10951,#10947,#1062,.T.);
#14348=EDGE_CURVE('',#10946,#10952,#1063,.T.);
#14349=EDGE_CURVE('',#10952,#10950,#1064,.T.);
#14350=EDGE_CURVE('',#10953,#10954,#6642,.T.);
#14351=EDGE_CURVE('',#10954,#10955,#1065,.T.);
#14352=EDGE_CURVE('',#10955,#10951,#1066,.T.);
#14353=EDGE_CURVE('',#10950,#10956,#1067,.T.);
#14354=EDGE_CURVE('',#10956,#10953,#1068,.T.);
#14355=EDGE_CURVE('',#10957,#10958,#6643,.T.);
#14356=EDGE_CURVE('',#10958,#10954,#1069,.T.);
#14357=EDGE_CURVE('',#10953,#10957,#1070,.T.);
#14358=EDGE_CURVE('',#10959,#10960,#6644,.T.);
#14359=EDGE_CURVE('',#10959,#10961,#1071,.T.);
#14360=EDGE_CURVE('',#10962,#10961,#5724,.F.);
#14361=EDGE_CURVE('',#10962,#10960,#1072,.T.);
#14362=EDGE_CURVE('',#10960,#10963,#1073,.T.);
#14363=EDGE_CURVE('',#10963,#10958,#1074,.T.);
#14364=EDGE_CURVE('',#10957,#10964,#1075,.T.);
#14365=EDGE_CURVE('',#10964,#10959,#1076,.T.);
#14366=EDGE_CURVE('',#10870,#10965,#1077,.T.);
#14367=EDGE_CURVE('',#10965,#10868,#1078,.T.);
#14368=EDGE_CURVE('',#10867,#10966,#1079,.T.);
#14369=EDGE_CURVE('',#10966,#10869,#1080,.T.);
#14370=EDGE_CURVE('',#10780,#10967,#1081,.T.);
#14371=EDGE_CURVE('',#10967,#10778,#1082,.T.);
#14372=EDGE_CURVE('',#10777,#10968,#1083,.T.);
#14373=EDGE_CURVE('',#10968,#10779,#1084,.T.);
#14374=EDGE_CURVE('',#10690,#10969,#1085,.T.);
#14375=EDGE_CURVE('',#10969,#10688,#1086,.T.);
#14376=EDGE_CURVE('',#10687,#10970,#1087,.T.);
#14377=EDGE_CURVE('',#10970,#10689,#1088,.T.);
#14378=EDGE_CURVE('',#10599,#10971,#1089,.T.);
#14379=EDGE_CURVE('',#10971,#10595,#1090,.T.);
#14380=EDGE_CURVE('',#10594,#10972,#1091,.T.);
#14381=EDGE_CURVE('',#10972,#10598,#1092,.F.);
#14382=EDGE_CURVE('',#10586,#10582,#1093,.T.);
#14383=EDGE_CURVE('',#10581,#10973,#1094,.T.);
#14384=EDGE_CURVE('',#10585,#10973,#5725,.F.);
#14385=EDGE_CURVE('',#10567,#10974,#1095,.T.);
#14386=EDGE_CURVE('',#10974,#10563,#1096,.T.);
#14387=EDGE_CURVE('',#10975,#10562,#1097,.T.);
#14388=EDGE_CURVE('',#10566,#10975,#1098,.T.);
#14389=EDGE_CURVE('',#10455,#10976,#1099,.T.);
#14390=EDGE_CURVE('',#10976,#10451,#1100,.T.);
#14391=EDGE_CURVE('',#10977,#10450,#1101,.T.);
#14392=EDGE_CURVE('',#10454,#10977,#1102,.T.);
#14393=EDGE_CURVE('',#10343,#10978,#1103,.T.);
#14394=EDGE_CURVE('',#10978,#10339,#1104,.T.);
#14395=EDGE_CURVE('',#10979,#10338,#1105,.T.);
#14396=EDGE_CURVE('',#10342,#10979,#1106,.T.);
#14397=EDGE_CURVE('',#10231,#10980,#1107,.T.);
#14398=EDGE_CURVE('',#10980,#10227,#1108,.T.);
#14399=EDGE_CURVE('',#10981,#10226,#1109,.T.);
#14400=EDGE_CURVE('',#10230,#10981,#1110,.T.);
#14401=EDGE_CURVE('',#10119,#10982,#1111,.T.);
#14402=EDGE_CURVE('',#10982,#10115,#1112,.T.);
#14403=EDGE_CURVE('',#10983,#10114,#1113,.T.);
#14404=EDGE_CURVE('',#10118,#10983,#1114,.T.);
#14405=EDGE_CURVE('',#10101,#10984,#1115,.T.);
#14406=EDGE_CURVE('',#10984,#10097,#1116,.T.);
#14407=EDGE_CURVE('',#10985,#10096,#1117,.T.);
#14408=EDGE_CURVE('',#10100,#10985,#1118,.T.);
#14409=EDGE_CURVE('',#10986,#10986,#5726,.T.);
#14410=EDGE_CURVE('',#10986,#10987,#6645,.T.);
#14411=EDGE_CURVE('',#10987,#10987,#5727,.T.);
#14412=EDGE_CURVE('',#10988,#10989,#5728,.T.);
#14413=EDGE_CURVE('',#10990,#10988,#6646,.T.);
#14414=EDGE_CURVE('',#10990,#10991,#5729,.T.);
#14415=EDGE_CURVE('',#10989,#10991,#6647,.T.);
#14416=EDGE_CURVE('',#10991,#10992,#6648,.T.);
#14417=EDGE_CURVE('',#10993,#10990,#6649,.T.);
#14418=EDGE_CURVE('',#10994,#10993,#6650,.T.);
#14419=EDGE_CURVE('',#10992,#10994,#5730,.T.);
#14420=EDGE_CURVE('',#10995,#10995,#5731,.T.);
#14421=EDGE_CURVE('',#10995,#10996,#6651,.T.);
#14422=EDGE_CURVE('',#10996,#10996,#5732,.T.);
#14423=EDGE_CURVE('',#10997,#10998,#5733,.T.);
#14424=EDGE_CURVE('',#10999,#10997,#6652,.T.);
#14425=EDGE_CURVE('',#10999,#11000,#5734,.T.);
#14426=EDGE_CURVE('',#10998,#11000,#6653,.T.);
#14427=EDGE_CURVE('',#11001,#11002,#6654,.T.);
#14428=EDGE_CURVE('',#11000,#11001,#6655,.T.);
#14429=EDGE_CURVE('',#11003,#10999,#6656,.T.);
#14430=EDGE_CURVE('',#11002,#11003,#5735,.T.);
#14431=EDGE_CURVE('',#11004,#11004,#5736,.T.);
#14432=EDGE_CURVE('',#11004,#11005,#6657,.T.);
#14433=EDGE_CURVE('',#11005,#11005,#5737,.T.);
#14434=EDGE_CURVE('',#11006,#10993,#6658,.T.);
#14435=EDGE_CURVE('',#11006,#11007,#6659,.T.);
#14436=EDGE_CURVE('',#11007,#10994,#6660,.T.);
#14437=EDGE_CURVE('',#11008,#10997,#6661,.T.);
#14438=EDGE_CURVE('',#11009,#11008,#6662,.T.);
#14439=EDGE_CURVE('',#11010,#11009,#6663,.T.);
#14440=EDGE_CURVE('',#11010,#11003,#6664,.T.);
#14441=EDGE_CURVE('',#10998,#10988,#6665,.T.);
#14442=EDGE_CURVE('',#11011,#11001,#6666,.T.);
#14443=EDGE_CURVE('',#11006,#11011,#6667,.T.);
#14444=EDGE_CURVE('',#10989,#11012,#6668,.T.);
#14445=EDGE_CURVE('',#11012,#11013,#5738,.T.);
#14446=EDGE_CURVE('',#11013,#11014,#6669,.T.);
#14447=EDGE_CURVE('',#11014,#11015,#5739,.T.);
#14448=EDGE_CURVE('',#11015,#11016,#6670,.T.);
#14449=EDGE_CURVE('',#11016,#11017,#5740,.T.);
#14450=EDGE_CURVE('',#11017,#11018,#6671,.T.);
#14451=EDGE_CURVE('',#11018,#11019,#5741,.T.);
#14452=EDGE_CURVE('',#11019,#11020,#6672,.T.);
#14453=EDGE_CURVE('',#11020,#11021,#6673,.T.);
#14454=EDGE_CURVE('',#11021,#11022,#6674,.T.);
#14455=EDGE_CURVE('',#11022,#11023,#6675,.T.);
#14456=EDGE_CURVE('',#11023,#11024,#6676,.T.);
#14457=EDGE_CURVE('',#11024,#11025,#5742,.T.);
#14458=EDGE_CURVE('',#11025,#11026,#6677,.T.);
#14459=EDGE_CURVE('',#11026,#11027,#5743,.T.);
#14460=EDGE_CURVE('',#11027,#11028,#6678,.T.);
#14461=EDGE_CURVE('',#11028,#11029,#6679,.T.);
#14462=EDGE_CURVE('',#11029,#11030,#6680,.T.);
#14463=EDGE_CURVE('',#11030,#11031,#6681,.T.);
#14464=EDGE_CURVE('',#11031,#11032,#6682,.T.);
#14465=EDGE_CURVE('',#11032,#11033,#5744,.T.);
#14466=EDGE_CURVE('',#11033,#11034,#6683,.T.);
#14467=EDGE_CURVE('',#11034,#11035,#5745,.T.);
#14468=EDGE_CURVE('',#11035,#11036,#6684,.T.);
#14469=EDGE_CURVE('',#11036,#11037,#5746,.T.);
#14470=EDGE_CURVE('',#11037,#11038,#6685,.T.);
#14471=EDGE_CURVE('',#11038,#11008,#5747,.T.);
#14472=EDGE_CURVE('',#11039,#11039,#5748,.T.);
#14473=EDGE_CURVE('',#11040,#11040,#5749,.T.);
#14474=EDGE_CURVE('',#10876,#10128,#1119,.T.);
#14475=EDGE_CURVE('',#10127,#10877,#1120,.T.);
#14476=EDGE_CURVE('',#10786,#10240,#1121,.T.);
#14477=EDGE_CURVE('',#10239,#10787,#1122,.T.);
#14478=EDGE_CURVE('',#10696,#10352,#1123,.T.);
#14479=EDGE_CURVE('',#10351,#10697,#1124,.T.);
#14480=EDGE_CURVE('',#10606,#10464,#1125,.T.);
#14481=EDGE_CURVE('',#10463,#10607,#1126,.T.);
#14482=EDGE_CURVE('',#10090,#10590,#1127,.T.);
#14483=EDGE_CURVE('',#10600,#10104,#1128,.T.);
#14484=EDGE_CURVE('',#10593,#10091,#1129,.T.);
#14485=EDGE_CURVE('',#10103,#10601,#1130,.T.);
#14486=EDGE_CURVE('',#10108,#10587,#1131,.T.);
#14487=EDGE_CURVE('',#10574,#10122,#1132,.T.);
#14488=EDGE_CURVE('',#10973,#10109,#1133,.T.);
#14489=EDGE_CURVE('',#10121,#10575,#1134,.T.);
#14490=EDGE_CURVE('',#10961,#10234,#1135,.T.);
#14491=EDGE_CURVE('',#10233,#10962,#1136,.T.);
#14492=EDGE_CURVE('',#10871,#10346,#1137,.T.);
#14493=EDGE_CURVE('',#10345,#10872,#1138,.T.);
#14494=EDGE_CURVE('',#10781,#10458,#1139,.T.);
#14495=EDGE_CURVE('',#10457,#10782,#1140,.T.);
#14496=EDGE_CURVE('',#10691,#10570,#1141,.T.);
#14497=EDGE_CURVE('',#10569,#10692,#1142,.T.);
#14498=EDGE_CURVE('',#11041,#11042,#6686,.T.);
#14499=EDGE_CURVE('',#11041,#11043,#6687,.T.);
#14500=EDGE_CURVE('',#11044,#11043,#6688,.T.);
#14501=EDGE_CURVE('',#11042,#11044,#6689,.T.);
#14502=EDGE_CURVE('',#11042,#11045,#6690,.T.);
#14503=EDGE_CURVE('',#11046,#11044,#6691,.T.);
#14504=EDGE_CURVE('',#11045,#11046,#6692,.T.);
#14505=EDGE_CURVE('',#11045,#11047,#6693,.T.);
#14506=EDGE_CURVE('',#11048,#11046,#6694,.T.);
#14507=EDGE_CURVE('',#11047,#11048,#6695,.T.);
#14508=EDGE_CURVE('',#11047,#11049,#6696,.T.);
#14509=EDGE_CURVE('',#11050,#11048,#6697,.T.);
#14510=EDGE_CURVE('',#11049,#11050,#6698,.T.);
#14511=EDGE_CURVE('',#11049,#11051,#6699,.T.);
#14512=EDGE_CURVE('',#11052,#11050,#6700,.T.);
#14513=EDGE_CURVE('',#11051,#11052,#6701,.T.);
#14514=EDGE_CURVE('',#11051,#11053,#6702,.T.);
#14515=EDGE_CURVE('',#11054,#11052,#6703,.T.);
#14516=EDGE_CURVE('',#11053,#11054,#6704,.T.);
#14517=EDGE_CURVE('',#11053,#11041,#6705,.T.);
#14518=EDGE_CURVE('',#11043,#11054,#6706,.T.);
#14519=EDGE_CURVE('',#11055,#11055,#5750,.T.);
#14520=EDGE_CURVE('',#11055,#11056,#6707,.T.);
#14521=EDGE_CURVE('',#11056,#11056,#5751,.T.);
#14522=EDGE_CURVE('',#11057,#11058,#5752,.T.);
#14523=EDGE_CURVE('',#11057,#11059,#6708,.T.);
#14524=EDGE_CURVE('',#11060,#11059,#5753,.T.);
#14525=EDGE_CURVE('',#11058,#11060,#6709,.T.);
#14526=EDGE_CURVE('',#11058,#11061,#6710,.T.);
#14527=EDGE_CURVE('',#11062,#11060,#6711,.T.);
#14528=EDGE_CURVE('',#11061,#11062,#6712,.T.);
#14529=EDGE_CURVE('',#11061,#11063,#5754,.T.);
#14530=EDGE_CURVE('',#11064,#11062,#5755,.T.);
#14531=EDGE_CURVE('',#11063,#11064,#6713,.T.);
#14532=EDGE_CURVE('',#11063,#11020,#6714,.T.);
#14533=EDGE_CURVE('',#11021,#11064,#6715,.T.);
#14534=EDGE_CURVE('',#11023,#11057,#6716,.T.);
#14535=EDGE_CURVE('',#11059,#11022,#6717,.T.);
#14536=EDGE_CURVE('',#11065,#11065,#5756,.T.);
#14537=EDGE_CURVE('',#11066,#11066,#5757,.T.);
#14538=EDGE_CURVE('',#11067,#11068,#6718,.T.);
#14539=EDGE_CURVE('',#11067,#11069,#6719,.T.);
#14540=EDGE_CURVE('',#11070,#11069,#6720,.T.);
#14541=EDGE_CURVE('',#11068,#11070,#6721,.T.);
#14542=EDGE_CURVE('',#11068,#11071,#6722,.T.);
#14543=EDGE_CURVE('',#11072,#11070,#6723,.T.);
#14544=EDGE_CURVE('',#11071,#11072,#6724,.T.);
#14545=EDGE_CURVE('',#11071,#11073,#6725,.T.);
#14546=EDGE_CURVE('',#11074,#11072,#6726,.T.);
#14547=EDGE_CURVE('',#11073,#11074,#6727,.T.);
#14548=EDGE_CURVE('',#11073,#11075,#6728,.T.);
#14549=EDGE_CURVE('',#11076,#11074,#6729,.T.);
#14550=EDGE_CURVE('',#11075,#11076,#6730,.T.);
#14551=EDGE_CURVE('',#11075,#11077,#6731,.T.);
#14552=EDGE_CURVE('',#11078,#11076,#6732,.T.);
#14553=EDGE_CURVE('',#11077,#11078,#6733,.T.);
#14554=EDGE_CURVE('',#11077,#11079,#6734,.T.);
#14555=EDGE_CURVE('',#11080,#11078,#6735,.T.);
#14556=EDGE_CURVE('',#11079,#11080,#6736,.T.);
#14557=EDGE_CURVE('',#11079,#11067,#6737,.T.);
#14558=EDGE_CURVE('',#11069,#11080,#6738,.T.);
#14559=EDGE_CURVE('',#11081,#11081,#5758,.T.);
#14560=EDGE_CURVE('',#11081,#11082,#6739,.T.);
#14561=EDGE_CURVE('',#11082,#11082,#5759,.T.);
#14562=EDGE_CURVE('',#11083,#11083,#5760,.T.);
#14563=EDGE_CURVE('',#11083,#11065,#6740,.T.);
#14564=EDGE_CURVE('',#11084,#11084,#5761,.T.);
#14565=EDGE_CURVE('',#11084,#11066,#6741,.T.);
#14566=EDGE_CURVE('',#11085,#11086,#5762,.T.);
#14567=EDGE_CURVE('',#11085,#11087,#6742,.T.);
#14568=EDGE_CURVE('',#11087,#11088,#5763,.T.);
#14569=EDGE_CURVE('',#11086,#11088,#6743,.T.);
#14570=EDGE_CURVE('',#11089,#11085,#6744,.T.);
#14571=EDGE_CURVE('',#11089,#11090,#6745,.T.);
#14572=EDGE_CURVE('',#11090,#11087,#6746,.T.);
#14573=EDGE_CURVE('',#11091,#11089,#5764,.T.);
#14574=EDGE_CURVE('',#11091,#11092,#6747,.T.);
#14575=EDGE_CURVE('',#11092,#11090,#5765,.T.);
#14576=EDGE_CURVE('',#11031,#11091,#6748,.T.);
#14577=EDGE_CURVE('',#11030,#11092,#6749,.T.);
#14578=EDGE_CURVE('',#11086,#11028,#6750,.T.);
#14579=EDGE_CURVE('',#11088,#11029,#6751,.T.);
#14580=EDGE_CURVE('',#11093,#11093,#5766,.T.);
#14581=EDGE_CURVE('',#11094,#11094,#5767,.T.);
#14582=EDGE_CURVE('',#11095,#11096,#6752,.T.);
#14583=EDGE_CURVE('',#11095,#11097,#6753,.T.);
#14584=EDGE_CURVE('',#11097,#11098,#6754,.T.);
#14585=EDGE_CURVE('',#11096,#11098,#6755,.T.);
#14586=EDGE_CURVE('',#11099,#11095,#6756,.T.);
#14587=EDGE_CURVE('',#11099,#11100,#6757,.T.);
#14588=EDGE_CURVE('',#11100,#11097,#6758,.T.);
#14589=EDGE_CURVE('',#11101,#11099,#6759,.T.);
#14590=EDGE_CURVE('',#11101,#11102,#6760,.T.);
#14591=EDGE_CURVE('',#11102,#11100,#6761,.T.);
#14592=EDGE_CURVE('',#11103,#11101,#6762,.T.);
#14593=EDGE_CURVE('',#11103,#11104,#6763,.T.);
#14594=EDGE_CURVE('',#11104,#11102,#6764,.T.);
#14595=EDGE_CURVE('',#11105,#11103,#6765,.T.);
#14596=EDGE_CURVE('',#11105,#11106,#6766,.T.);
#14597=EDGE_CURVE('',#11106,#11104,#6767,.T.);
#14598=EDGE_CURVE('',#11107,#11105,#6768,.T.);
#14599=EDGE_CURVE('',#11107,#11108,#6769,.T.);
#14600=EDGE_CURVE('',#11108,#11106,#6770,.T.);
#14601=EDGE_CURVE('',#11096,#11107,#6771,.T.);
#14602=EDGE_CURVE('',#11098,#11108,#6772,.T.);
#14603=EDGE_CURVE('',#11109,#11109,#5768,.T.);
#14604=EDGE_CURVE('',#11109,#11110,#6773,.T.);
#14605=EDGE_CURVE('',#11110,#11110,#5769,.T.);
#14606=EDGE_CURVE('',#11111,#11112,#6774,.T.);
#14607=EDGE_CURVE('',#11111,#11113,#6775,.T.);
#14608=EDGE_CURVE('',#11113,#11114,#6776,.T.);
#14609=EDGE_CURVE('',#11112,#11114,#6777,.T.);
#14610=EDGE_CURVE('',#11115,#11111,#6778,.T.);
#14611=EDGE_CURVE('',#11115,#11116,#6779,.T.);
#14612=EDGE_CURVE('',#11116,#11113,#6780,.T.);
#14613=EDGE_CURVE('',#11117,#11115,#6781,.T.);
#14614=EDGE_CURVE('',#11117,#11118,#6782,.T.);
#14615=EDGE_CURVE('',#11118,#11116,#6783,.T.);
#14616=EDGE_CURVE('',#11119,#11117,#6784,.T.);
#14617=EDGE_CURVE('',#11119,#11120,#6785,.T.);
#14618=EDGE_CURVE('',#11120,#11118,#6786,.T.);
#14619=EDGE_CURVE('',#11121,#11119,#6787,.T.);
#14620=EDGE_CURVE('',#11121,#11122,#6788,.T.);
#14621=EDGE_CURVE('',#11122,#11120,#6789,.T.);
#14622=EDGE_CURVE('',#11123,#11121,#6790,.T.);
#14623=EDGE_CURVE('',#11123,#11124,#6791,.T.);
#14624=EDGE_CURVE('',#11124,#11122,#6792,.T.);
#14625=EDGE_CURVE('',#11112,#11123,#6793,.T.);
#14626=EDGE_CURVE('',#11114,#11124,#6794,.T.);
#14627=EDGE_CURVE('',#11125,#11125,#5770,.T.);
#14628=EDGE_CURVE('',#11125,#11126,#6795,.T.);
#14629=EDGE_CURVE('',#11126,#11126,#5771,.T.);
#14630=EDGE_CURVE('',#11127,#11027,#6796,.T.);
#14631=EDGE_CURVE('',#11128,#11127,#6797,.T.);
#14632=EDGE_CURVE('',#11128,#11032,#6798,.T.);
#14633=EDGE_CURVE('',#11094,#11129,#6799,.T.);
#14634=EDGE_CURVE('',#11129,#11129,#5772,.T.);
#14635=EDGE_CURVE('',#11093,#11130,#6800,.T.);
#14636=EDGE_CURVE('',#11130,#11130,#5773,.T.);
#14637=EDGE_CURVE('',#11039,#11131,#6801,.T.);
#14638=EDGE_CURVE('',#11131,#11131,#5774,.T.);
#14639=EDGE_CURVE('',#11040,#11132,#6802,.T.);
#14640=EDGE_CURVE('',#11132,#11132,#5775,.T.);
#14641=EDGE_CURVE('',#11133,#11002,#6803,.T.);
#14642=EDGE_CURVE('',#11011,#11133,#6804,.T.);
#14643=EDGE_CURVE('',#11133,#11010,#5776,.T.);
#14644=EDGE_CURVE('',#11134,#11009,#5777,.T.);
#14645=EDGE_CURVE('',#11134,#11038,#6805,.T.);
#14646=EDGE_CURVE('',#11134,#11135,#6806,.T.);
#14647=EDGE_CURVE('',#11135,#11037,#6807,.T.);
#14648=EDGE_CURVE('',#11135,#11136,#5778,.T.);
#14649=EDGE_CURVE('',#11136,#11036,#6808,.T.);
#14650=EDGE_CURVE('',#11136,#11137,#6809,.T.);
#14651=EDGE_CURVE('',#11137,#11035,#6810,.T.);
#14652=EDGE_CURVE('',#11137,#11138,#5779,.T.);
#14653=EDGE_CURVE('',#11138,#11034,#6811,.T.);
#14654=EDGE_CURVE('',#11138,#11139,#6812,.T.);
#14655=EDGE_CURVE('',#11139,#11033,#6813,.T.);
#14656=EDGE_CURVE('',#11139,#11128,#5780,.T.);
#14657=EDGE_CURVE('',#11127,#11140,#5781,.T.);
#14658=EDGE_CURVE('',#11140,#11026,#6814,.T.);
#14659=EDGE_CURVE('',#11140,#11141,#6815,.T.);
#14660=EDGE_CURVE('',#11141,#11025,#6816,.T.);
#14661=EDGE_CURVE('',#11141,#11142,#5782,.T.);
#14662=EDGE_CURVE('',#11142,#11024,#6817,.T.);
#14663=EDGE_CURVE('',#11143,#11019,#6818,.T.);
#14664=EDGE_CURVE('',#11143,#11142,#6819,.T.);
#14665=EDGE_CURVE('',#11143,#11144,#5783,.T.);
#14666=EDGE_CURVE('',#11144,#11018,#6820,.T.);
#14667=EDGE_CURVE('',#11145,#11144,#6821,.T.);
#14668=EDGE_CURVE('',#11145,#11017,#6822,.T.);
#14669=EDGE_CURVE('',#11145,#11146,#5784,.T.);
#14670=EDGE_CURVE('',#11146,#11016,#6823,.T.);
#14671=EDGE_CURVE('',#11147,#11146,#6824,.T.);
#14672=EDGE_CURVE('',#11147,#11015,#6825,.T.);
#14673=EDGE_CURVE('',#11147,#11148,#5785,.T.);
#14674=EDGE_CURVE('',#11148,#11014,#6826,.T.);
#14675=EDGE_CURVE('',#11149,#11148,#6827,.T.);
#14676=EDGE_CURVE('',#11149,#11013,#6828,.T.);
#14677=EDGE_CURVE('',#11150,#11149,#5786,.T.);
#14678=EDGE_CURVE('',#11150,#11012,#6829,.T.);
#14679=EDGE_CURVE('',#11151,#10992,#6830,.T.);
#14680=EDGE_CURVE('',#11151,#11150,#6831,.T.);
#14681=EDGE_CURVE('',#11151,#11007,#5787,.T.);
#17835=ORIENTED_EDGE('',*,*,#13279,.T.);
#17836=ORIENTED_EDGE('',*,*,#13280,.T.);
#17837=ORIENTED_EDGE('',*,*,#13281,.F.);
#17838=ORIENTED_EDGE('',*,*,#13282,.F.);
#17839=ORIENTED_EDGE('',*,*,#13283,.T.);
#17840=ORIENTED_EDGE('',*,*,#13284,.T.);
#17841=ORIENTED_EDGE('',*,*,#13285,.T.);
#17842=ORIENTED_EDGE('',*,*,#13279,.F.);
#17843=ORIENTED_EDGE('',*,*,#13286,.F.);
#17844=ORIENTED_EDGE('',*,*,#13287,.F.);
#17845=ORIENTED_EDGE('',*,*,#13288,.T.);
#17846=ORIENTED_EDGE('',*,*,#13289,.T.);
#17847=ORIENTED_EDGE('',*,*,#13290,.T.);
#17848=ORIENTED_EDGE('',*,*,#13283,.F.);
#17849=ORIENTED_EDGE('',*,*,#13291,.F.);
#17850=ORIENTED_EDGE('',*,*,#13292,.F.);
#17851=ORIENTED_EDGE('',*,*,#13293,.F.);
#17852=ORIENTED_EDGE('',*,*,#13294,.F.);
#17853=ORIENTED_EDGE('',*,*,#13295,.F.);
#17854=ORIENTED_EDGE('',*,*,#13296,.F.);
#17855=ORIENTED_EDGE('',*,*,#13297,.T.);
#17856=ORIENTED_EDGE('',*,*,#13298,.T.);
#17857=ORIENTED_EDGE('',*,*,#13299,.T.);
#17858=ORIENTED_EDGE('',*,*,#13300,.T.);
#17859=ORIENTED_EDGE('',*,*,#13301,.F.);
#17860=ORIENTED_EDGE('',*,*,#13302,.F.);
#17861=ORIENTED_EDGE('',*,*,#13303,.T.);
#17862=ORIENTED_EDGE('',*,*,#13304,.T.);
#17863=ORIENTED_EDGE('',*,*,#13305,.T.);
#17864=ORIENTED_EDGE('',*,*,#13299,.F.);
#17865=ORIENTED_EDGE('',*,*,#13306,.F.);
#17866=ORIENTED_EDGE('',*,*,#13307,.F.);
#17867=ORIENTED_EDGE('',*,*,#13308,.T.);
#17868=ORIENTED_EDGE('',*,*,#13309,.T.);
#17869=ORIENTED_EDGE('',*,*,#13310,.T.);
#17870=ORIENTED_EDGE('',*,*,#13303,.F.);
#17871=ORIENTED_EDGE('',*,*,#13311,.F.);
#17872=ORIENTED_EDGE('',*,*,#13312,.F.);
#17873=ORIENTED_EDGE('',*,*,#13313,.F.);
#17874=ORIENTED_EDGE('',*,*,#13314,.F.);
#17875=ORIENTED_EDGE('',*,*,#13315,.F.);
#17876=ORIENTED_EDGE('',*,*,#13316,.F.);
#17877=ORIENTED_EDGE('',*,*,#13317,.T.);
#17878=ORIENTED_EDGE('',*,*,#13318,.T.);
#17879=ORIENTED_EDGE('',*,*,#13319,.T.);
#17880=ORIENTED_EDGE('',*,*,#13320,.T.);
#17881=ORIENTED_EDGE('',*,*,#13321,.T.);
#17882=ORIENTED_EDGE('',*,*,#13322,.F.);
#17883=ORIENTED_EDGE('',*,*,#13323,.F.);
#17884=ORIENTED_EDGE('',*,*,#13324,.F.);
#17885=ORIENTED_EDGE('',*,*,#13325,.T.);
#17886=ORIENTED_EDGE('',*,*,#13326,.T.);
#17887=ORIENTED_EDGE('',*,*,#13327,.T.);
#17888=ORIENTED_EDGE('',*,*,#13319,.F.);
#17889=ORIENTED_EDGE('',*,*,#13328,.F.);
#17890=ORIENTED_EDGE('',*,*,#13329,.F.);
#17891=ORIENTED_EDGE('',*,*,#13330,.T.);
#17892=ORIENTED_EDGE('',*,*,#13331,.T.);
#17893=ORIENTED_EDGE('',*,*,#13332,.T.);
#17894=ORIENTED_EDGE('',*,*,#13325,.F.);
#17895=ORIENTED_EDGE('',*,*,#13333,.F.);
#17896=ORIENTED_EDGE('',*,*,#13334,.F.);
#17897=ORIENTED_EDGE('',*,*,#13335,.T.);
#17898=ORIENTED_EDGE('',*,*,#13336,.T.);
#17899=ORIENTED_EDGE('',*,*,#13337,.T.);
#17900=ORIENTED_EDGE('',*,*,#13330,.F.);
#17901=ORIENTED_EDGE('',*,*,#13338,.F.);
#17902=ORIENTED_EDGE('',*,*,#13339,.F.);
#17903=ORIENTED_EDGE('',*,*,#13340,.T.);
#17904=ORIENTED_EDGE('',*,*,#13341,.T.);
#17905=ORIENTED_EDGE('',*,*,#13342,.T.);
#17906=ORIENTED_EDGE('',*,*,#13335,.F.);
#17907=ORIENTED_EDGE('',*,*,#13343,.F.);
#17908=ORIENTED_EDGE('',*,*,#13344,.F.);
#17909=ORIENTED_EDGE('',*,*,#13345,.T.);
#17910=ORIENTED_EDGE('',*,*,#13346,.T.);
#17911=ORIENTED_EDGE('',*,*,#13347,.T.);
#17912=ORIENTED_EDGE('',*,*,#13340,.F.);
#17913=ORIENTED_EDGE('',*,*,#13348,.F.);
#17914=ORIENTED_EDGE('',*,*,#13349,.F.);
#17915=ORIENTED_EDGE('',*,*,#13350,.T.);
#17916=ORIENTED_EDGE('',*,*,#13351,.T.);
#17917=ORIENTED_EDGE('',*,*,#13352,.T.);
#17918=ORIENTED_EDGE('',*,*,#13345,.F.);
#17919=ORIENTED_EDGE('',*,*,#13353,.F.);
#17920=ORIENTED_EDGE('',*,*,#13354,.F.);
#17921=ORIENTED_EDGE('',*,*,#13355,.T.);
#17922=ORIENTED_EDGE('',*,*,#13356,.T.);
#17923=ORIENTED_EDGE('',*,*,#13357,.T.);
#17924=ORIENTED_EDGE('',*,*,#13350,.F.);
#17925=ORIENTED_EDGE('',*,*,#13358,.F.);
#17926=ORIENTED_EDGE('',*,*,#13359,.F.);
#17927=ORIENTED_EDGE('',*,*,#13360,.T.);
#17928=ORIENTED_EDGE('',*,*,#13361,.T.);
#17929=ORIENTED_EDGE('',*,*,#13362,.T.);
#17930=ORIENTED_EDGE('',*,*,#13355,.F.);
#17931=ORIENTED_EDGE('',*,*,#13363,.F.);
#17932=ORIENTED_EDGE('',*,*,#13364,.F.);
#17933=ORIENTED_EDGE('',*,*,#13365,.T.);
#17934=ORIENTED_EDGE('',*,*,#13366,.T.);
#17935=ORIENTED_EDGE('',*,*,#13367,.T.);
#17936=ORIENTED_EDGE('',*,*,#13360,.F.);
#17937=ORIENTED_EDGE('',*,*,#13368,.F.);
#17938=ORIENTED_EDGE('',*,*,#13369,.F.);
#17939=ORIENTED_EDGE('',*,*,#13370,.T.);
#17940=ORIENTED_EDGE('',*,*,#13371,.T.);
#17941=ORIENTED_EDGE('',*,*,#13372,.T.);
#17942=ORIENTED_EDGE('',*,*,#13365,.F.);
#17943=ORIENTED_EDGE('',*,*,#13373,.F.);
#17944=ORIENTED_EDGE('',*,*,#13374,.F.);
#17945=ORIENTED_EDGE('',*,*,#13375,.T.);
#17946=ORIENTED_EDGE('',*,*,#13376,.T.);
#17947=ORIENTED_EDGE('',*,*,#13377,.T.);
#17948=ORIENTED_EDGE('',*,*,#13370,.F.);
#17949=ORIENTED_EDGE('',*,*,#13378,.F.);
#17950=ORIENTED_EDGE('',*,*,#13379,.F.);
#17951=ORIENTED_EDGE('',*,*,#13380,.T.);
#17952=ORIENTED_EDGE('',*,*,#13381,.T.);
#17953=ORIENTED_EDGE('',*,*,#13382,.T.);
#17954=ORIENTED_EDGE('',*,*,#13375,.F.);
#17955=ORIENTED_EDGE('',*,*,#13383,.F.);
#17956=ORIENTED_EDGE('',*,*,#13384,.F.);
#17957=ORIENTED_EDGE('',*,*,#13385,.T.);
#17958=ORIENTED_EDGE('',*,*,#13386,.T.);
#17959=ORIENTED_EDGE('',*,*,#13387,.T.);
#17960=ORIENTED_EDGE('',*,*,#13380,.F.);
#17961=ORIENTED_EDGE('',*,*,#13388,.F.);
#17962=ORIENTED_EDGE('',*,*,#13389,.F.);
#17963=ORIENTED_EDGE('',*,*,#13390,.T.);
#17964=ORIENTED_EDGE('',*,*,#13391,.T.);
#17965=ORIENTED_EDGE('',*,*,#13392,.T.);
#17966=ORIENTED_EDGE('',*,*,#13385,.F.);
#17967=ORIENTED_EDGE('',*,*,#13393,.F.);
#17968=ORIENTED_EDGE('',*,*,#13394,.F.);
#17969=ORIENTED_EDGE('',*,*,#13395,.T.);
#17970=ORIENTED_EDGE('',*,*,#13396,.T.);
#17971=ORIENTED_EDGE('',*,*,#13397,.T.);
#17972=ORIENTED_EDGE('',*,*,#13390,.F.);
#17973=ORIENTED_EDGE('',*,*,#13398,.F.);
#17974=ORIENTED_EDGE('',*,*,#13399,.F.);
#17975=ORIENTED_EDGE('',*,*,#13400,.T.);
#17976=ORIENTED_EDGE('',*,*,#13401,.T.);
#17977=ORIENTED_EDGE('',*,*,#13402,.T.);
#17978=ORIENTED_EDGE('',*,*,#13395,.F.);
#17979=ORIENTED_EDGE('',*,*,#13403,.F.);
#17980=ORIENTED_EDGE('',*,*,#13404,.F.);
#17981=ORIENTED_EDGE('',*,*,#13405,.T.);
#17982=ORIENTED_EDGE('',*,*,#13406,.T.);
#17983=ORIENTED_EDGE('',*,*,#13407,.T.);
#17984=ORIENTED_EDGE('',*,*,#13400,.F.);
#17985=ORIENTED_EDGE('',*,*,#13408,.F.);
#17986=ORIENTED_EDGE('',*,*,#13409,.F.);
#17987=ORIENTED_EDGE('',*,*,#13410,.T.);
#17988=ORIENTED_EDGE('',*,*,#13411,.T.);
#17989=ORIENTED_EDGE('',*,*,#13412,.T.);
#17990=ORIENTED_EDGE('',*,*,#13405,.F.);
#17991=ORIENTED_EDGE('',*,*,#13413,.F.);
#17992=ORIENTED_EDGE('',*,*,#13414,.F.);
#17993=ORIENTED_EDGE('',*,*,#13415,.T.);
#17994=ORIENTED_EDGE('',*,*,#13416,.T.);
#17995=ORIENTED_EDGE('',*,*,#13417,.T.);
#17996=ORIENTED_EDGE('',*,*,#13410,.F.);
#17997=ORIENTED_EDGE('',*,*,#13418,.F.);
#17998=ORIENTED_EDGE('',*,*,#13419,.F.);
#17999=ORIENTED_EDGE('',*,*,#13420,.T.);
#18000=ORIENTED_EDGE('',*,*,#13421,.T.);
#18001=ORIENTED_EDGE('',*,*,#13422,.T.);
#18002=ORIENTED_EDGE('',*,*,#13415,.F.);
#18003=ORIENTED_EDGE('',*,*,#13423,.F.);
#18004=ORIENTED_EDGE('',*,*,#13424,.F.);
#18005=ORIENTED_EDGE('',*,*,#13425,.T.);
#18006=ORIENTED_EDGE('',*,*,#13426,.T.);
#18007=ORIENTED_EDGE('',*,*,#13427,.T.);
#18008=ORIENTED_EDGE('',*,*,#13420,.F.);
#18009=ORIENTED_EDGE('',*,*,#13428,.F.);
#18010=ORIENTED_EDGE('',*,*,#13429,.F.);
#18011=ORIENTED_EDGE('',*,*,#13430,.T.);
#18012=ORIENTED_EDGE('',*,*,#13431,.T.);
#18013=ORIENTED_EDGE('',*,*,#13432,.T.);
#18014=ORIENTED_EDGE('',*,*,#13425,.F.);
#18015=ORIENTED_EDGE('',*,*,#13433,.F.);
#18016=ORIENTED_EDGE('',*,*,#13434,.F.);
#18017=ORIENTED_EDGE('',*,*,#13435,.T.);
#18018=ORIENTED_EDGE('',*,*,#13436,.T.);
#18019=ORIENTED_EDGE('',*,*,#13437,.T.);
#18020=ORIENTED_EDGE('',*,*,#13430,.F.);
#18021=ORIENTED_EDGE('',*,*,#13438,.F.);
#18022=ORIENTED_EDGE('',*,*,#13439,.F.);
#18023=ORIENTED_EDGE('',*,*,#13440,.T.);
#18024=ORIENTED_EDGE('',*,*,#13441,.T.);
#18025=ORIENTED_EDGE('',*,*,#13442,.T.);
#18026=ORIENTED_EDGE('',*,*,#13435,.F.);
#18027=ORIENTED_EDGE('',*,*,#13443,.F.);
#18028=ORIENTED_EDGE('',*,*,#13444,.F.);
#18029=ORIENTED_EDGE('',*,*,#13445,.T.);
#18030=ORIENTED_EDGE('',*,*,#13446,.T.);
#18031=ORIENTED_EDGE('',*,*,#13447,.T.);
#18032=ORIENTED_EDGE('',*,*,#13440,.F.);
#18033=ORIENTED_EDGE('',*,*,#13448,.F.);
#18034=ORIENTED_EDGE('',*,*,#13449,.F.);
#18035=ORIENTED_EDGE('',*,*,#13450,.F.);
#18036=ORIENTED_EDGE('',*,*,#13451,.F.);
#18037=ORIENTED_EDGE('',*,*,#13452,.F.);
#18038=ORIENTED_EDGE('',*,*,#13453,.F.);
#18039=ORIENTED_EDGE('',*,*,#13454,.T.);
#18040=ORIENTED_EDGE('',*,*,#13455,.T.);
#18041=ORIENTED_EDGE('',*,*,#13456,.T.);
#18042=ORIENTED_EDGE('',*,*,#13457,.T.);
#18043=ORIENTED_EDGE('',*,*,#13458,.T.);
#18044=ORIENTED_EDGE('',*,*,#13459,.F.);
#18045=ORIENTED_EDGE('',*,*,#13460,.F.);
#18046=ORIENTED_EDGE('',*,*,#13461,.F.);
#18047=ORIENTED_EDGE('',*,*,#13462,.T.);
#18048=ORIENTED_EDGE('',*,*,#13463,.T.);
#18049=ORIENTED_EDGE('',*,*,#13464,.T.);
#18050=ORIENTED_EDGE('',*,*,#13456,.F.);
#18051=ORIENTED_EDGE('',*,*,#13465,.F.);
#18052=ORIENTED_EDGE('',*,*,#13466,.F.);
#18053=ORIENTED_EDGE('',*,*,#13467,.T.);
#18054=ORIENTED_EDGE('',*,*,#13468,.T.);
#18055=ORIENTED_EDGE('',*,*,#13469,.T.);
#18056=ORIENTED_EDGE('',*,*,#13462,.F.);
#18057=ORIENTED_EDGE('',*,*,#13470,.F.);
#18058=ORIENTED_EDGE('',*,*,#13471,.F.);
#18059=ORIENTED_EDGE('',*,*,#13472,.T.);
#18060=ORIENTED_EDGE('',*,*,#13473,.T.);
#18061=ORIENTED_EDGE('',*,*,#13474,.T.);
#18062=ORIENTED_EDGE('',*,*,#13467,.F.);
#18063=ORIENTED_EDGE('',*,*,#13475,.F.);
#18064=ORIENTED_EDGE('',*,*,#13476,.F.);
#18065=ORIENTED_EDGE('',*,*,#13477,.T.);
#18066=ORIENTED_EDGE('',*,*,#13478,.T.);
#18067=ORIENTED_EDGE('',*,*,#13479,.T.);
#18068=ORIENTED_EDGE('',*,*,#13472,.F.);
#18069=ORIENTED_EDGE('',*,*,#13480,.F.);
#18070=ORIENTED_EDGE('',*,*,#13481,.F.);
#18071=ORIENTED_EDGE('',*,*,#13482,.T.);
#18072=ORIENTED_EDGE('',*,*,#13483,.T.);
#18073=ORIENTED_EDGE('',*,*,#13484,.T.);
#18074=ORIENTED_EDGE('',*,*,#13477,.F.);
#18075=ORIENTED_EDGE('',*,*,#13485,.F.);
#18076=ORIENTED_EDGE('',*,*,#13486,.F.);
#18077=ORIENTED_EDGE('',*,*,#13487,.T.);
#18078=ORIENTED_EDGE('',*,*,#13488,.T.);
#18079=ORIENTED_EDGE('',*,*,#13489,.T.);
#18080=ORIENTED_EDGE('',*,*,#13482,.F.);
#18081=ORIENTED_EDGE('',*,*,#13490,.F.);
#18082=ORIENTED_EDGE('',*,*,#13491,.F.);
#18083=ORIENTED_EDGE('',*,*,#13492,.T.);
#18084=ORIENTED_EDGE('',*,*,#13493,.T.);
#18085=ORIENTED_EDGE('',*,*,#13494,.T.);
#18086=ORIENTED_EDGE('',*,*,#13487,.F.);
#18087=ORIENTED_EDGE('',*,*,#13495,.F.);
#18088=ORIENTED_EDGE('',*,*,#13496,.F.);
#18089=ORIENTED_EDGE('',*,*,#13497,.T.);
#18090=ORIENTED_EDGE('',*,*,#13498,.T.);
#18091=ORIENTED_EDGE('',*,*,#13499,.T.);
#18092=ORIENTED_EDGE('',*,*,#13492,.F.);
#18093=ORIENTED_EDGE('',*,*,#13500,.F.);
#18094=ORIENTED_EDGE('',*,*,#13501,.F.);
#18095=ORIENTED_EDGE('',*,*,#13502,.T.);
#18096=ORIENTED_EDGE('',*,*,#13503,.T.);
#18097=ORIENTED_EDGE('',*,*,#13504,.T.);
#18098=ORIENTED_EDGE('',*,*,#13497,.F.);
#18099=ORIENTED_EDGE('',*,*,#13505,.F.);
#18100=ORIENTED_EDGE('',*,*,#13506,.F.);
#18101=ORIENTED_EDGE('',*,*,#13507,.T.);
#18102=ORIENTED_EDGE('',*,*,#13508,.T.);
#18103=ORIENTED_EDGE('',*,*,#13509,.T.);
#18104=ORIENTED_EDGE('',*,*,#13502,.F.);
#18105=ORIENTED_EDGE('',*,*,#13510,.F.);
#18106=ORIENTED_EDGE('',*,*,#13511,.F.);
#18107=ORIENTED_EDGE('',*,*,#13512,.T.);
#18108=ORIENTED_EDGE('',*,*,#13513,.T.);
#18109=ORIENTED_EDGE('',*,*,#13514,.T.);
#18110=ORIENTED_EDGE('',*,*,#13507,.F.);
#18111=ORIENTED_EDGE('',*,*,#13515,.F.);
#18112=ORIENTED_EDGE('',*,*,#13516,.F.);
#18113=ORIENTED_EDGE('',*,*,#13517,.T.);
#18114=ORIENTED_EDGE('',*,*,#13518,.T.);
#18115=ORIENTED_EDGE('',*,*,#13519,.T.);
#18116=ORIENTED_EDGE('',*,*,#13512,.F.);
#18117=ORIENTED_EDGE('',*,*,#13520,.F.);
#18118=ORIENTED_EDGE('',*,*,#13521,.F.);
#18119=ORIENTED_EDGE('',*,*,#13522,.T.);
#18120=ORIENTED_EDGE('',*,*,#13523,.T.);
#18121=ORIENTED_EDGE('',*,*,#13524,.T.);
#18122=ORIENTED_EDGE('',*,*,#13517,.F.);
#18123=ORIENTED_EDGE('',*,*,#13525,.F.);
#18124=ORIENTED_EDGE('',*,*,#13526,.F.);
#18125=ORIENTED_EDGE('',*,*,#13527,.T.);
#18126=ORIENTED_EDGE('',*,*,#13528,.T.);
#18127=ORIENTED_EDGE('',*,*,#13529,.T.);
#18128=ORIENTED_EDGE('',*,*,#13522,.F.);
#18129=ORIENTED_EDGE('',*,*,#13530,.F.);
#18130=ORIENTED_EDGE('',*,*,#13531,.F.);
#18131=ORIENTED_EDGE('',*,*,#13532,.T.);
#18132=ORIENTED_EDGE('',*,*,#13533,.T.);
#18133=ORIENTED_EDGE('',*,*,#13534,.T.);
#18134=ORIENTED_EDGE('',*,*,#13527,.F.);
#18135=ORIENTED_EDGE('',*,*,#13535,.F.);
#18136=ORIENTED_EDGE('',*,*,#13536,.F.);
#18137=ORIENTED_EDGE('',*,*,#13537,.T.);
#18138=ORIENTED_EDGE('',*,*,#13538,.T.);
#18139=ORIENTED_EDGE('',*,*,#13539,.T.);
#18140=ORIENTED_EDGE('',*,*,#13532,.F.);
#18141=ORIENTED_EDGE('',*,*,#13540,.F.);
#18142=ORIENTED_EDGE('',*,*,#13541,.F.);
#18143=ORIENTED_EDGE('',*,*,#13542,.T.);
#18144=ORIENTED_EDGE('',*,*,#13543,.T.);
#18145=ORIENTED_EDGE('',*,*,#13544,.T.);
#18146=ORIENTED_EDGE('',*,*,#13537,.F.);
#18147=ORIENTED_EDGE('',*,*,#13545,.F.);
#18148=ORIENTED_EDGE('',*,*,#13546,.F.);
#18149=ORIENTED_EDGE('',*,*,#13547,.T.);
#18150=ORIENTED_EDGE('',*,*,#13548,.T.);
#18151=ORIENTED_EDGE('',*,*,#13549,.T.);
#18152=ORIENTED_EDGE('',*,*,#13542,.F.);
#18153=ORIENTED_EDGE('',*,*,#13550,.F.);
#18154=ORIENTED_EDGE('',*,*,#13551,.F.);
#18155=ORIENTED_EDGE('',*,*,#13552,.T.);
#18156=ORIENTED_EDGE('',*,*,#13553,.T.);
#18157=ORIENTED_EDGE('',*,*,#13554,.T.);
#18158=ORIENTED_EDGE('',*,*,#13547,.F.);
#18159=ORIENTED_EDGE('',*,*,#13555,.F.);
#18160=ORIENTED_EDGE('',*,*,#13556,.F.);
#18161=ORIENTED_EDGE('',*,*,#13557,.T.);
#18162=ORIENTED_EDGE('',*,*,#13558,.T.);
#18163=ORIENTED_EDGE('',*,*,#13559,.T.);
#18164=ORIENTED_EDGE('',*,*,#13552,.F.);
#18165=ORIENTED_EDGE('',*,*,#13560,.F.);
#18166=ORIENTED_EDGE('',*,*,#13561,.F.);
#18167=ORIENTED_EDGE('',*,*,#13562,.T.);
#18168=ORIENTED_EDGE('',*,*,#13563,.T.);
#18169=ORIENTED_EDGE('',*,*,#13564,.T.);
#18170=ORIENTED_EDGE('',*,*,#13557,.F.);
#18171=ORIENTED_EDGE('',*,*,#13565,.F.);
#18172=ORIENTED_EDGE('',*,*,#13566,.F.);
#18173=ORIENTED_EDGE('',*,*,#13567,.T.);
#18174=ORIENTED_EDGE('',*,*,#13568,.T.);
#18175=ORIENTED_EDGE('',*,*,#13569,.T.);
#18176=ORIENTED_EDGE('',*,*,#13562,.F.);
#18177=ORIENTED_EDGE('',*,*,#13570,.F.);
#18178=ORIENTED_EDGE('',*,*,#13571,.F.);
#18179=ORIENTED_EDGE('',*,*,#13572,.T.);
#18180=ORIENTED_EDGE('',*,*,#13573,.T.);
#18181=ORIENTED_EDGE('',*,*,#13574,.T.);
#18182=ORIENTED_EDGE('',*,*,#13567,.F.);
#18183=ORIENTED_EDGE('',*,*,#13575,.F.);
#18184=ORIENTED_EDGE('',*,*,#13576,.F.);
#18185=ORIENTED_EDGE('',*,*,#13577,.T.);
#18186=ORIENTED_EDGE('',*,*,#13578,.T.);
#18187=ORIENTED_EDGE('',*,*,#13579,.T.);
#18188=ORIENTED_EDGE('',*,*,#13572,.F.);
#18189=ORIENTED_EDGE('',*,*,#13580,.F.);
#18190=ORIENTED_EDGE('',*,*,#13581,.F.);
#18191=ORIENTED_EDGE('',*,*,#13582,.T.);
#18192=ORIENTED_EDGE('',*,*,#13583,.T.);
#18193=ORIENTED_EDGE('',*,*,#13584,.T.);
#18194=ORIENTED_EDGE('',*,*,#13577,.F.);
#18195=ORIENTED_EDGE('',*,*,#13585,.F.);
#18196=ORIENTED_EDGE('',*,*,#13586,.F.);
#18197=ORIENTED_EDGE('',*,*,#13587,.F.);
#18198=ORIENTED_EDGE('',*,*,#13588,.F.);
#18199=ORIENTED_EDGE('',*,*,#13589,.F.);
#18200=ORIENTED_EDGE('',*,*,#13590,.F.);
#18201=ORIENTED_EDGE('',*,*,#13591,.T.);
#18202=ORIENTED_EDGE('',*,*,#13592,.T.);
#18203=ORIENTED_EDGE('',*,*,#13593,.T.);
#18204=ORIENTED_EDGE('',*,*,#13594,.T.);
#18205=ORIENTED_EDGE('',*,*,#13595,.T.);
#18206=ORIENTED_EDGE('',*,*,#13596,.F.);
#18207=ORIENTED_EDGE('',*,*,#13597,.F.);
#18208=ORIENTED_EDGE('',*,*,#13598,.F.);
#18209=ORIENTED_EDGE('',*,*,#13599,.T.);
#18210=ORIENTED_EDGE('',*,*,#13600,.T.);
#18211=ORIENTED_EDGE('',*,*,#13601,.T.);
#18212=ORIENTED_EDGE('',*,*,#13593,.F.);
#18213=ORIENTED_EDGE('',*,*,#13602,.F.);
#18214=ORIENTED_EDGE('',*,*,#13603,.F.);
#18215=ORIENTED_EDGE('',*,*,#13604,.T.);
#18216=ORIENTED_EDGE('',*,*,#13605,.T.);
#18217=ORIENTED_EDGE('',*,*,#13606,.T.);
#18218=ORIENTED_EDGE('',*,*,#13599,.F.);
#18219=ORIENTED_EDGE('',*,*,#13607,.F.);
#18220=ORIENTED_EDGE('',*,*,#13608,.F.);
#18221=ORIENTED_EDGE('',*,*,#13609,.T.);
#18222=ORIENTED_EDGE('',*,*,#13610,.T.);
#18223=ORIENTED_EDGE('',*,*,#13611,.T.);
#18224=ORIENTED_EDGE('',*,*,#13604,.F.);
#18225=ORIENTED_EDGE('',*,*,#13612,.F.);
#18226=ORIENTED_EDGE('',*,*,#13613,.F.);
#18227=ORIENTED_EDGE('',*,*,#13614,.T.);
#18228=ORIENTED_EDGE('',*,*,#13615,.T.);
#18229=ORIENTED_EDGE('',*,*,#13616,.T.);
#18230=ORIENTED_EDGE('',*,*,#13609,.F.);
#18231=ORIENTED_EDGE('',*,*,#13617,.F.);
#18232=ORIENTED_EDGE('',*,*,#13618,.F.);
#18233=ORIENTED_EDGE('',*,*,#13619,.T.);
#18234=ORIENTED_EDGE('',*,*,#13620,.T.);
#18235=ORIENTED_EDGE('',*,*,#13621,.T.);
#18236=ORIENTED_EDGE('',*,*,#13614,.F.);
#18237=ORIENTED_EDGE('',*,*,#13622,.F.);
#18238=ORIENTED_EDGE('',*,*,#13623,.F.);
#18239=ORIENTED_EDGE('',*,*,#13624,.T.);
#18240=ORIENTED_EDGE('',*,*,#13625,.T.);
#18241=ORIENTED_EDGE('',*,*,#13626,.T.);
#18242=ORIENTED_EDGE('',*,*,#13619,.F.);
#18243=ORIENTED_EDGE('',*,*,#13627,.F.);
#18244=ORIENTED_EDGE('',*,*,#13628,.F.);
#18245=ORIENTED_EDGE('',*,*,#13629,.T.);
#18246=ORIENTED_EDGE('',*,*,#13630,.T.);
#18247=ORIENTED_EDGE('',*,*,#13631,.T.);
#18248=ORIENTED_EDGE('',*,*,#13624,.F.);
#18249=ORIENTED_EDGE('',*,*,#13632,.F.);
#18250=ORIENTED_EDGE('',*,*,#13633,.F.);
#18251=ORIENTED_EDGE('',*,*,#13634,.T.);
#18252=ORIENTED_EDGE('',*,*,#13635,.T.);
#18253=ORIENTED_EDGE('',*,*,#13636,.T.);
#18254=ORIENTED_EDGE('',*,*,#13629,.F.);
#18255=ORIENTED_EDGE('',*,*,#13637,.F.);
#18256=ORIENTED_EDGE('',*,*,#13638,.F.);
#18257=ORIENTED_EDGE('',*,*,#13639,.T.);
#18258=ORIENTED_EDGE('',*,*,#13640,.T.);
#18259=ORIENTED_EDGE('',*,*,#13641,.T.);
#18260=ORIENTED_EDGE('',*,*,#13634,.F.);
#18261=ORIENTED_EDGE('',*,*,#13642,.F.);
#18262=ORIENTED_EDGE('',*,*,#13643,.F.);
#18263=ORIENTED_EDGE('',*,*,#13644,.T.);
#18264=ORIENTED_EDGE('',*,*,#13645,.T.);
#18265=ORIENTED_EDGE('',*,*,#13646,.T.);
#18266=ORIENTED_EDGE('',*,*,#13639,.F.);
#18267=ORIENTED_EDGE('',*,*,#13647,.F.);
#18268=ORIENTED_EDGE('',*,*,#13648,.F.);
#18269=ORIENTED_EDGE('',*,*,#13649,.T.);
#18270=ORIENTED_EDGE('',*,*,#13650,.T.);
#18271=ORIENTED_EDGE('',*,*,#13651,.T.);
#18272=ORIENTED_EDGE('',*,*,#13644,.F.);
#18273=ORIENTED_EDGE('',*,*,#13652,.F.);
#18274=ORIENTED_EDGE('',*,*,#13653,.F.);
#18275=ORIENTED_EDGE('',*,*,#13654,.T.);
#18276=ORIENTED_EDGE('',*,*,#13655,.T.);
#18277=ORIENTED_EDGE('',*,*,#13656,.T.);
#18278=ORIENTED_EDGE('',*,*,#13649,.F.);
#18279=ORIENTED_EDGE('',*,*,#13657,.F.);
#18280=ORIENTED_EDGE('',*,*,#13658,.F.);
#18281=ORIENTED_EDGE('',*,*,#13659,.T.);
#18282=ORIENTED_EDGE('',*,*,#13660,.T.);
#18283=ORIENTED_EDGE('',*,*,#13661,.T.);
#18284=ORIENTED_EDGE('',*,*,#13654,.F.);
#18285=ORIENTED_EDGE('',*,*,#13662,.F.);
#18286=ORIENTED_EDGE('',*,*,#13663,.F.);
#18287=ORIENTED_EDGE('',*,*,#13664,.T.);
#18288=ORIENTED_EDGE('',*,*,#13665,.T.);
#18289=ORIENTED_EDGE('',*,*,#13666,.T.);
#18290=ORIENTED_EDGE('',*,*,#13659,.F.);
#18291=ORIENTED_EDGE('',*,*,#13667,.F.);
#18292=ORIENTED_EDGE('',*,*,#13668,.F.);
#18293=ORIENTED_EDGE('',*,*,#13669,.T.);
#18294=ORIENTED_EDGE('',*,*,#13670,.T.);
#18295=ORIENTED_EDGE('',*,*,#13671,.T.);
#18296=ORIENTED_EDGE('',*,*,#13664,.F.);
#18297=ORIENTED_EDGE('',*,*,#13672,.F.);
#18298=ORIENTED_EDGE('',*,*,#13673,.F.);
#18299=ORIENTED_EDGE('',*,*,#13674,.T.);
#18300=ORIENTED_EDGE('',*,*,#13675,.T.);
#18301=ORIENTED_EDGE('',*,*,#13676,.T.);
#18302=ORIENTED_EDGE('',*,*,#13669,.F.);
#18303=ORIENTED_EDGE('',*,*,#13677,.F.);
#18304=ORIENTED_EDGE('',*,*,#13678,.F.);
#18305=ORIENTED_EDGE('',*,*,#13679,.T.);
#18306=ORIENTED_EDGE('',*,*,#13680,.T.);
#18307=ORIENTED_EDGE('',*,*,#13681,.T.);
#18308=ORIENTED_EDGE('',*,*,#13674,.F.);
#18309=ORIENTED_EDGE('',*,*,#13682,.F.);
#18310=ORIENTED_EDGE('',*,*,#13683,.F.);
#18311=ORIENTED_EDGE('',*,*,#13684,.T.);
#18312=ORIENTED_EDGE('',*,*,#13685,.T.);
#18313=ORIENTED_EDGE('',*,*,#13686,.T.);
#18314=ORIENTED_EDGE('',*,*,#13679,.F.);
#18315=ORIENTED_EDGE('',*,*,#13687,.F.);
#18316=ORIENTED_EDGE('',*,*,#13688,.F.);
#18317=ORIENTED_EDGE('',*,*,#13689,.T.);
#18318=ORIENTED_EDGE('',*,*,#13690,.T.);
#18319=ORIENTED_EDGE('',*,*,#13691,.T.);
#18320=ORIENTED_EDGE('',*,*,#13684,.F.);
#18321=ORIENTED_EDGE('',*,*,#13692,.F.);
#18322=ORIENTED_EDGE('',*,*,#13693,.F.);
#18323=ORIENTED_EDGE('',*,*,#13694,.T.);
#18324=ORIENTED_EDGE('',*,*,#13695,.T.);
#18325=ORIENTED_EDGE('',*,*,#13696,.T.);
#18326=ORIENTED_EDGE('',*,*,#13689,.F.);
#18327=ORIENTED_EDGE('',*,*,#13697,.F.);
#18328=ORIENTED_EDGE('',*,*,#13698,.F.);
#18329=ORIENTED_EDGE('',*,*,#13699,.T.);
#18330=ORIENTED_EDGE('',*,*,#13700,.T.);
#18331=ORIENTED_EDGE('',*,*,#13701,.T.);
#18332=ORIENTED_EDGE('',*,*,#13694,.F.);
#18333=ORIENTED_EDGE('',*,*,#13702,.F.);
#18334=ORIENTED_EDGE('',*,*,#13703,.F.);
#18335=ORIENTED_EDGE('',*,*,#13704,.T.);
#18336=ORIENTED_EDGE('',*,*,#13705,.T.);
#18337=ORIENTED_EDGE('',*,*,#13706,.T.);
#18338=ORIENTED_EDGE('',*,*,#13699,.F.);
#18339=ORIENTED_EDGE('',*,*,#13707,.F.);
#18340=ORIENTED_EDGE('',*,*,#13708,.F.);
#18341=ORIENTED_EDGE('',*,*,#13709,.T.);
#18342=ORIENTED_EDGE('',*,*,#13710,.T.);
#18343=ORIENTED_EDGE('',*,*,#13711,.T.);
#18344=ORIENTED_EDGE('',*,*,#13704,.F.);
#18345=ORIENTED_EDGE('',*,*,#13712,.F.);
#18346=ORIENTED_EDGE('',*,*,#13713,.F.);
#18347=ORIENTED_EDGE('',*,*,#13714,.T.);
#18348=ORIENTED_EDGE('',*,*,#13715,.T.);
#18349=ORIENTED_EDGE('',*,*,#13716,.T.);
#18350=ORIENTED_EDGE('',*,*,#13709,.F.);
#18351=ORIENTED_EDGE('',*,*,#13717,.F.);
#18352=ORIENTED_EDGE('',*,*,#13718,.F.);
#18353=ORIENTED_EDGE('',*,*,#13719,.T.);
#18354=ORIENTED_EDGE('',*,*,#13720,.T.);
#18355=ORIENTED_EDGE('',*,*,#13721,.T.);
#18356=ORIENTED_EDGE('',*,*,#13714,.F.);
#18357=ORIENTED_EDGE('',*,*,#13722,.F.);
#18358=ORIENTED_EDGE('',*,*,#13723,.F.);
#18359=ORIENTED_EDGE('',*,*,#13724,.F.);
#18360=ORIENTED_EDGE('',*,*,#13725,.F.);
#18361=ORIENTED_EDGE('',*,*,#13726,.F.);
#18362=ORIENTED_EDGE('',*,*,#13727,.F.);
#18363=ORIENTED_EDGE('',*,*,#13728,.T.);
#18364=ORIENTED_EDGE('',*,*,#13729,.T.);
#18365=ORIENTED_EDGE('',*,*,#13730,.T.);
#18366=ORIENTED_EDGE('',*,*,#13731,.T.);
#18367=ORIENTED_EDGE('',*,*,#13732,.T.);
#18368=ORIENTED_EDGE('',*,*,#13733,.F.);
#18369=ORIENTED_EDGE('',*,*,#13734,.F.);
#18370=ORIENTED_EDGE('',*,*,#13735,.F.);
#18371=ORIENTED_EDGE('',*,*,#13736,.T.);
#18372=ORIENTED_EDGE('',*,*,#13737,.T.);
#18373=ORIENTED_EDGE('',*,*,#13738,.T.);
#18374=ORIENTED_EDGE('',*,*,#13730,.F.);
#18375=ORIENTED_EDGE('',*,*,#13739,.F.);
#18376=ORIENTED_EDGE('',*,*,#13740,.F.);
#18377=ORIENTED_EDGE('',*,*,#13741,.T.);
#18378=ORIENTED_EDGE('',*,*,#13742,.T.);
#18379=ORIENTED_EDGE('',*,*,#13743,.T.);
#18380=ORIENTED_EDGE('',*,*,#13736,.F.);
#18381=ORIENTED_EDGE('',*,*,#13744,.F.);
#18382=ORIENTED_EDGE('',*,*,#13745,.F.);
#18383=ORIENTED_EDGE('',*,*,#13746,.T.);
#18384=ORIENTED_EDGE('',*,*,#13747,.T.);
#18385=ORIENTED_EDGE('',*,*,#13748,.T.);
#18386=ORIENTED_EDGE('',*,*,#13741,.F.);
#18387=ORIENTED_EDGE('',*,*,#13749,.F.);
#18388=ORIENTED_EDGE('',*,*,#13750,.F.);
#18389=ORIENTED_EDGE('',*,*,#13751,.T.);
#18390=ORIENTED_EDGE('',*,*,#13752,.T.);
#18391=ORIENTED_EDGE('',*,*,#13753,.T.);
#18392=ORIENTED_EDGE('',*,*,#13746,.F.);
#18393=ORIENTED_EDGE('',*,*,#13754,.F.);
#18394=ORIENTED_EDGE('',*,*,#13755,.F.);
#18395=ORIENTED_EDGE('',*,*,#13756,.T.);
#18396=ORIENTED_EDGE('',*,*,#13757,.T.);
#18397=ORIENTED_EDGE('',*,*,#13758,.T.);
#18398=ORIENTED_EDGE('',*,*,#13751,.F.);
#18399=ORIENTED_EDGE('',*,*,#13759,.F.);
#18400=ORIENTED_EDGE('',*,*,#13760,.F.);
#18401=ORIENTED_EDGE('',*,*,#13761,.T.);
#18402=ORIENTED_EDGE('',*,*,#13762,.T.);
#18403=ORIENTED_EDGE('',*,*,#13763,.T.);
#18404=ORIENTED_EDGE('',*,*,#13756,.F.);
#18405=ORIENTED_EDGE('',*,*,#13764,.F.);
#18406=ORIENTED_EDGE('',*,*,#13765,.F.);
#18407=ORIENTED_EDGE('',*,*,#13766,.T.);
#18408=ORIENTED_EDGE('',*,*,#13767,.T.);
#18409=ORIENTED_EDGE('',*,*,#13768,.T.);
#18410=ORIENTED_EDGE('',*,*,#13761,.F.);
#18411=ORIENTED_EDGE('',*,*,#13769,.F.);
#18412=ORIENTED_EDGE('',*,*,#13770,.F.);
#18413=ORIENTED_EDGE('',*,*,#13771,.T.);
#18414=ORIENTED_EDGE('',*,*,#13772,.T.);
#18415=ORIENTED_EDGE('',*,*,#13773,.T.);
#18416=ORIENTED_EDGE('',*,*,#13766,.F.);
#18417=ORIENTED_EDGE('',*,*,#13774,.F.);
#18418=ORIENTED_EDGE('',*,*,#13775,.F.);
#18419=ORIENTED_EDGE('',*,*,#13776,.T.);
#18420=ORIENTED_EDGE('',*,*,#13777,.T.);
#18421=ORIENTED_EDGE('',*,*,#13778,.T.);
#18422=ORIENTED_EDGE('',*,*,#13771,.F.);
#18423=ORIENTED_EDGE('',*,*,#13779,.F.);
#18424=ORIENTED_EDGE('',*,*,#13780,.F.);
#18425=ORIENTED_EDGE('',*,*,#13781,.T.);
#18426=ORIENTED_EDGE('',*,*,#13782,.T.);
#18427=ORIENTED_EDGE('',*,*,#13783,.T.);
#18428=ORIENTED_EDGE('',*,*,#13776,.F.);
#18429=ORIENTED_EDGE('',*,*,#13784,.F.);
#18430=ORIENTED_EDGE('',*,*,#13785,.F.);
#18431=ORIENTED_EDGE('',*,*,#13786,.T.);
#18432=ORIENTED_EDGE('',*,*,#13787,.T.);
#18433=ORIENTED_EDGE('',*,*,#13788,.T.);
#18434=ORIENTED_EDGE('',*,*,#13781,.F.);
#18435=ORIENTED_EDGE('',*,*,#13789,.F.);
#18436=ORIENTED_EDGE('',*,*,#13790,.F.);
#18437=ORIENTED_EDGE('',*,*,#13791,.T.);
#18438=ORIENTED_EDGE('',*,*,#13792,.T.);
#18439=ORIENTED_EDGE('',*,*,#13793,.T.);
#18440=ORIENTED_EDGE('',*,*,#13786,.F.);
#18441=ORIENTED_EDGE('',*,*,#13794,.F.);
#18442=ORIENTED_EDGE('',*,*,#13795,.F.);
#18443=ORIENTED_EDGE('',*,*,#13796,.T.);
#18444=ORIENTED_EDGE('',*,*,#13797,.T.);
#18445=ORIENTED_EDGE('',*,*,#13798,.T.);
#18446=ORIENTED_EDGE('',*,*,#13791,.F.);
#18447=ORIENTED_EDGE('',*,*,#13799,.F.);
#18448=ORIENTED_EDGE('',*,*,#13800,.F.);
#18449=ORIENTED_EDGE('',*,*,#13801,.T.);
#18450=ORIENTED_EDGE('',*,*,#13802,.T.);
#18451=ORIENTED_EDGE('',*,*,#13803,.T.);
#18452=ORIENTED_EDGE('',*,*,#13796,.F.);
#18453=ORIENTED_EDGE('',*,*,#13804,.F.);
#18454=ORIENTED_EDGE('',*,*,#13805,.F.);
#18455=ORIENTED_EDGE('',*,*,#13806,.T.);
#18456=ORIENTED_EDGE('',*,*,#13807,.T.);
#18457=ORIENTED_EDGE('',*,*,#13808,.T.);
#18458=ORIENTED_EDGE('',*,*,#13801,.F.);
#18459=ORIENTED_EDGE('',*,*,#13809,.F.);
#18460=ORIENTED_EDGE('',*,*,#13810,.F.);
#18461=ORIENTED_EDGE('',*,*,#13811,.T.);
#18462=ORIENTED_EDGE('',*,*,#13812,.T.);
#18463=ORIENTED_EDGE('',*,*,#13813,.T.);
#18464=ORIENTED_EDGE('',*,*,#13806,.F.);
#18465=ORIENTED_EDGE('',*,*,#13814,.F.);
#18466=ORIENTED_EDGE('',*,*,#13815,.F.);
#18467=ORIENTED_EDGE('',*,*,#13816,.T.);
#18468=ORIENTED_EDGE('',*,*,#13817,.T.);
#18469=ORIENTED_EDGE('',*,*,#13818,.T.);
#18470=ORIENTED_EDGE('',*,*,#13811,.F.);
#18471=ORIENTED_EDGE('',*,*,#13819,.F.);
#18472=ORIENTED_EDGE('',*,*,#13820,.F.);
#18473=ORIENTED_EDGE('',*,*,#13821,.T.);
#18474=ORIENTED_EDGE('',*,*,#13822,.T.);
#18475=ORIENTED_EDGE('',*,*,#13823,.T.);
#18476=ORIENTED_EDGE('',*,*,#13816,.F.);
#18477=ORIENTED_EDGE('',*,*,#13824,.F.);
#18478=ORIENTED_EDGE('',*,*,#13825,.F.);
#18479=ORIENTED_EDGE('',*,*,#13826,.T.);
#18480=ORIENTED_EDGE('',*,*,#13827,.T.);
#18481=ORIENTED_EDGE('',*,*,#13828,.T.);
#18482=ORIENTED_EDGE('',*,*,#13821,.F.);
#18483=ORIENTED_EDGE('',*,*,#13829,.F.);
#18484=ORIENTED_EDGE('',*,*,#13830,.F.);
#18485=ORIENTED_EDGE('',*,*,#13831,.T.);
#18486=ORIENTED_EDGE('',*,*,#13832,.T.);
#18487=ORIENTED_EDGE('',*,*,#13833,.T.);
#18488=ORIENTED_EDGE('',*,*,#13826,.F.);
#18489=ORIENTED_EDGE('',*,*,#13834,.F.);
#18490=ORIENTED_EDGE('',*,*,#13835,.F.);
#18491=ORIENTED_EDGE('',*,*,#13836,.T.);
#18492=ORIENTED_EDGE('',*,*,#13837,.T.);
#18493=ORIENTED_EDGE('',*,*,#13838,.T.);
#18494=ORIENTED_EDGE('',*,*,#13831,.F.);
#18495=ORIENTED_EDGE('',*,*,#13839,.F.);
#18496=ORIENTED_EDGE('',*,*,#13840,.F.);
#18497=ORIENTED_EDGE('',*,*,#13841,.T.);
#18498=ORIENTED_EDGE('',*,*,#13842,.T.);
#18499=ORIENTED_EDGE('',*,*,#13843,.T.);
#18500=ORIENTED_EDGE('',*,*,#13836,.F.);
#18501=ORIENTED_EDGE('',*,*,#13844,.F.);
#18502=ORIENTED_EDGE('',*,*,#13845,.F.);
#18503=ORIENTED_EDGE('',*,*,#13846,.T.);
#18504=ORIENTED_EDGE('',*,*,#13847,.T.);
#18505=ORIENTED_EDGE('',*,*,#13848,.T.);
#18506=ORIENTED_EDGE('',*,*,#13841,.F.);
#18507=ORIENTED_EDGE('',*,*,#13849,.F.);
#18508=ORIENTED_EDGE('',*,*,#13850,.F.);
#18509=ORIENTED_EDGE('',*,*,#13851,.T.);
#18510=ORIENTED_EDGE('',*,*,#13852,.T.);
#18511=ORIENTED_EDGE('',*,*,#13853,.T.);
#18512=ORIENTED_EDGE('',*,*,#13846,.F.);
#18513=ORIENTED_EDGE('',*,*,#13854,.F.);
#18514=ORIENTED_EDGE('',*,*,#13855,.F.);
#18515=ORIENTED_EDGE('',*,*,#13856,.T.);
#18516=ORIENTED_EDGE('',*,*,#13857,.T.);
#18517=ORIENTED_EDGE('',*,*,#13858,.T.);
#18518=ORIENTED_EDGE('',*,*,#13851,.F.);
#18519=ORIENTED_EDGE('',*,*,#13859,.F.);
#18520=ORIENTED_EDGE('',*,*,#13860,.F.);
#18521=ORIENTED_EDGE('',*,*,#13861,.F.);
#18522=ORIENTED_EDGE('',*,*,#13862,.F.);
#18523=ORIENTED_EDGE('',*,*,#13863,.F.);
#18524=ORIENTED_EDGE('',*,*,#13864,.F.);
#18525=ORIENTED_EDGE('',*,*,#13865,.T.);
#18526=ORIENTED_EDGE('',*,*,#13866,.T.);
#18527=ORIENTED_EDGE('',*,*,#13867,.T.);
#18528=ORIENTED_EDGE('',*,*,#13868,.T.);
#18529=ORIENTED_EDGE('',*,*,#13869,.T.);
#18530=ORIENTED_EDGE('',*,*,#13870,.T.);
#18531=ORIENTED_EDGE('',*,*,#13871,.T.);
#18532=ORIENTED_EDGE('',*,*,#13872,.T.);
#18533=ORIENTED_EDGE('',*,*,#13873,.T.);
#18534=ORIENTED_EDGE('',*,*,#13874,.T.);
#18535=ORIENTED_EDGE('',*,*,#13867,.F.);
#18536=ORIENTED_EDGE('',*,*,#13875,.T.);
#18537=ORIENTED_EDGE('',*,*,#13876,.T.);
#18538=ORIENTED_EDGE('',*,*,#13877,.T.);
#18539=ORIENTED_EDGE('',*,*,#13878,.T.);
#18540=ORIENTED_EDGE('',*,*,#13879,.T.);
#18541=ORIENTED_EDGE('',*,*,#13872,.F.);
#18542=ORIENTED_EDGE('',*,*,#13880,.T.);
#18543=ORIENTED_EDGE('',*,*,#13881,.T.);
#18544=ORIENTED_EDGE('',*,*,#13882,.F.);
#18545=ORIENTED_EDGE('',*,*,#13883,.F.);
#18546=ORIENTED_EDGE('',*,*,#13884,.T.);
#18547=ORIENTED_EDGE('',*,*,#13885,.T.);
#18548=ORIENTED_EDGE('',*,*,#13886,.T.);
#18549=ORIENTED_EDGE('',*,*,#13887,.T.);
#18550=ORIENTED_EDGE('',*,*,#13888,.T.);
#18551=ORIENTED_EDGE('',*,*,#13889,.T.);
#18552=ORIENTED_EDGE('',*,*,#13890,.T.);
#18553=ORIENTED_EDGE('',*,*,#13885,.F.);
#18554=ORIENTED_EDGE('',*,*,#13891,.T.);
#18555=ORIENTED_EDGE('',*,*,#13892,.T.);
#18556=ORIENTED_EDGE('',*,*,#13893,.T.);
#18557=ORIENTED_EDGE('',*,*,#13894,.T.);
#18558=ORIENTED_EDGE('',*,*,#13888,.F.);
#18559=ORIENTED_EDGE('',*,*,#13895,.T.);
#18560=ORIENTED_EDGE('',*,*,#13896,.T.);
#18561=ORIENTED_EDGE('',*,*,#13897,.F.);
#18562=ORIENTED_EDGE('',*,*,#13898,.T.);
#18563=ORIENTED_EDGE('',*,*,#13899,.T.);
#18564=ORIENTED_EDGE('',*,*,#13900,.T.);
#18565=ORIENTED_EDGE('',*,*,#13901,.T.);
#18566=ORIENTED_EDGE('',*,*,#13902,.T.);
#18567=ORIENTED_EDGE('',*,*,#13903,.T.);
#18568=ORIENTED_EDGE('',*,*,#13904,.T.);
#18569=ORIENTED_EDGE('',*,*,#13905,.F.);
#18570=ORIENTED_EDGE('',*,*,#13906,.T.);
#18571=ORIENTED_EDGE('',*,*,#13907,.T.);
#18572=ORIENTED_EDGE('',*,*,#13908,.T.);
#18573=ORIENTED_EDGE('',*,*,#13909,.T.);
#18574=ORIENTED_EDGE('',*,*,#13902,.F.);
#18575=ORIENTED_EDGE('',*,*,#13910,.T.);
#18576=ORIENTED_EDGE('',*,*,#13911,.T.);
#18577=ORIENTED_EDGE('',*,*,#13912,.T.);
#18578=ORIENTED_EDGE('',*,*,#13913,.T.);
#18579=ORIENTED_EDGE('',*,*,#13908,.F.);
#18580=ORIENTED_EDGE('',*,*,#13914,.T.);
#18581=ORIENTED_EDGE('',*,*,#13915,.T.);
#18582=ORIENTED_EDGE('',*,*,#13916,.T.);
#18583=ORIENTED_EDGE('',*,*,#13917,.T.);
#18584=ORIENTED_EDGE('',*,*,#13918,.T.);
#18585=ORIENTED_EDGE('',*,*,#13911,.F.);
#18586=ORIENTED_EDGE('',*,*,#13919,.T.);
#18587=ORIENTED_EDGE('',*,*,#13920,.T.);
#18588=ORIENTED_EDGE('',*,*,#13921,.T.);
#18589=ORIENTED_EDGE('',*,*,#13922,.T.);
#18590=ORIENTED_EDGE('',*,*,#13916,.F.);
#18591=ORIENTED_EDGE('',*,*,#13923,.T.);
#18592=ORIENTED_EDGE('',*,*,#13924,.T.);
#18593=ORIENTED_EDGE('',*,*,#13925,.T.);
#18594=ORIENTED_EDGE('',*,*,#13926,.T.);
#18595=ORIENTED_EDGE('',*,*,#13920,.F.);
#18596=ORIENTED_EDGE('',*,*,#13927,.T.);
#18597=ORIENTED_EDGE('',*,*,#13928,.T.);
#18598=ORIENTED_EDGE('',*,*,#13929,.T.);
#18599=ORIENTED_EDGE('',*,*,#13930,.T.);
#18600=ORIENTED_EDGE('',*,*,#13925,.F.);
#18601=ORIENTED_EDGE('',*,*,#13931,.T.);
#18602=ORIENTED_EDGE('',*,*,#13932,.T.);
#18603=ORIENTED_EDGE('',*,*,#13933,.T.);
#18604=ORIENTED_EDGE('',*,*,#13934,.T.);
#18605=ORIENTED_EDGE('',*,*,#13928,.F.);
#18606=ORIENTED_EDGE('',*,*,#13935,.T.);
#18607=ORIENTED_EDGE('',*,*,#13936,.T.);
#18608=ORIENTED_EDGE('',*,*,#13937,.T.);
#18609=ORIENTED_EDGE('',*,*,#13938,.T.);
#18610=ORIENTED_EDGE('',*,*,#13933,.F.);
#18611=ORIENTED_EDGE('',*,*,#13939,.T.);
#18612=ORIENTED_EDGE('',*,*,#13940,.T.);
#18613=ORIENTED_EDGE('',*,*,#13941,.T.);
#18614=ORIENTED_EDGE('',*,*,#13942,.T.);
#18615=ORIENTED_EDGE('',*,*,#13943,.T.);
#18616=ORIENTED_EDGE('',*,*,#13936,.F.);
#18617=ORIENTED_EDGE('',*,*,#13944,.T.);
#18618=ORIENTED_EDGE('',*,*,#13945,.T.);
#18619=ORIENTED_EDGE('',*,*,#13946,.T.);
#18620=ORIENTED_EDGE('',*,*,#13947,.T.);
#18621=ORIENTED_EDGE('',*,*,#13941,.F.);
#18622=ORIENTED_EDGE('',*,*,#13948,.T.);
#18623=ORIENTED_EDGE('',*,*,#13949,.T.);
#18624=ORIENTED_EDGE('',*,*,#13950,.T.);
#18625=ORIENTED_EDGE('',*,*,#13951,.T.);
#18626=ORIENTED_EDGE('',*,*,#13945,.F.);
#18627=ORIENTED_EDGE('',*,*,#13952,.T.);
#18628=ORIENTED_EDGE('',*,*,#13953,.T.);
#18629=ORIENTED_EDGE('',*,*,#13954,.T.);
#18630=ORIENTED_EDGE('',*,*,#13955,.T.);
#18631=ORIENTED_EDGE('',*,*,#13956,.T.);
#18632=ORIENTED_EDGE('',*,*,#13950,.F.);
#18633=ORIENTED_EDGE('',*,*,#13957,.T.);
#18634=ORIENTED_EDGE('',*,*,#13958,.T.);
#18635=ORIENTED_EDGE('',*,*,#13959,.T.);
#18636=ORIENTED_EDGE('',*,*,#13960,.T.);
#18637=ORIENTED_EDGE('',*,*,#13954,.F.);
#18638=ORIENTED_EDGE('',*,*,#13961,.T.);
#18639=ORIENTED_EDGE('',*,*,#13962,.T.);
#18640=ORIENTED_EDGE('',*,*,#13963,.T.);
#18641=ORIENTED_EDGE('',*,*,#13964,.T.);
#18642=ORIENTED_EDGE('',*,*,#13959,.F.);
#18643=ORIENTED_EDGE('',*,*,#13965,.T.);
#18644=ORIENTED_EDGE('',*,*,#13966,.T.);
#18645=ORIENTED_EDGE('',*,*,#13967,.T.);
#18646=ORIENTED_EDGE('',*,*,#13968,.T.);
#18647=ORIENTED_EDGE('',*,*,#13969,.T.);
#18648=ORIENTED_EDGE('',*,*,#13962,.F.);
#18649=ORIENTED_EDGE('',*,*,#13970,.T.);
#18650=ORIENTED_EDGE('',*,*,#13971,.T.);
#18651=ORIENTED_EDGE('',*,*,#13972,.T.);
#18652=ORIENTED_EDGE('',*,*,#13973,.T.);
#18653=ORIENTED_EDGE('',*,*,#13967,.F.);
#18654=ORIENTED_EDGE('',*,*,#13974,.T.);
#18655=ORIENTED_EDGE('',*,*,#13975,.T.);
#18656=ORIENTED_EDGE('',*,*,#13976,.T.);
#18657=ORIENTED_EDGE('',*,*,#13977,.T.);
#18658=ORIENTED_EDGE('',*,*,#13971,.F.);
#18659=ORIENTED_EDGE('',*,*,#13978,.T.);
#18660=ORIENTED_EDGE('',*,*,#13979,.T.);
#18661=ORIENTED_EDGE('',*,*,#13980,.T.);
#18662=ORIENTED_EDGE('',*,*,#13981,.T.);
#18663=ORIENTED_EDGE('',*,*,#13982,.T.);
#18664=ORIENTED_EDGE('',*,*,#13976,.F.);
#18665=ORIENTED_EDGE('',*,*,#13983,.T.);
#18666=ORIENTED_EDGE('',*,*,#13984,.T.);
#18667=ORIENTED_EDGE('',*,*,#13985,.T.);
#18668=ORIENTED_EDGE('',*,*,#13986,.T.);
#18669=ORIENTED_EDGE('',*,*,#13980,.F.);
#18670=ORIENTED_EDGE('',*,*,#13987,.T.);
#18671=ORIENTED_EDGE('',*,*,#13988,.T.);
#18672=ORIENTED_EDGE('',*,*,#13989,.T.);
#18673=ORIENTED_EDGE('',*,*,#13990,.T.);
#18674=ORIENTED_EDGE('',*,*,#13985,.F.);
#18675=ORIENTED_EDGE('',*,*,#13991,.T.);
#18676=ORIENTED_EDGE('',*,*,#13992,.T.);
#18677=ORIENTED_EDGE('',*,*,#13993,.T.);
#18678=ORIENTED_EDGE('',*,*,#13994,.T.);
#18679=ORIENTED_EDGE('',*,*,#13988,.F.);
#18680=ORIENTED_EDGE('',*,*,#13995,.T.);
#18681=ORIENTED_EDGE('',*,*,#13996,.T.);
#18682=ORIENTED_EDGE('',*,*,#13997,.T.);
#18683=ORIENTED_EDGE('',*,*,#13998,.T.);
#18684=ORIENTED_EDGE('',*,*,#13993,.F.);
#18685=ORIENTED_EDGE('',*,*,#13999,.T.);
#18686=ORIENTED_EDGE('',*,*,#14000,.T.);
#18687=ORIENTED_EDGE('',*,*,#14001,.T.);
#18688=ORIENTED_EDGE('',*,*,#14002,.T.);
#18689=ORIENTED_EDGE('',*,*,#13996,.F.);
#18690=ORIENTED_EDGE('',*,*,#14003,.T.);
#18691=ORIENTED_EDGE('',*,*,#14004,.T.);
#18692=ORIENTED_EDGE('',*,*,#14005,.T.);
#18693=ORIENTED_EDGE('',*,*,#14006,.T.);
#18694=ORIENTED_EDGE('',*,*,#14007,.T.);
#18695=ORIENTED_EDGE('',*,*,#14001,.F.);
#18696=ORIENTED_EDGE('',*,*,#14008,.T.);
#18697=ORIENTED_EDGE('',*,*,#14009,.T.);
#18698=ORIENTED_EDGE('',*,*,#14010,.T.);
#18699=ORIENTED_EDGE('',*,*,#14011,.T.);
#18700=ORIENTED_EDGE('',*,*,#14005,.F.);
#18701=ORIENTED_EDGE('',*,*,#14012,.T.);
#18702=ORIENTED_EDGE('',*,*,#14013,.F.);
#18703=ORIENTED_EDGE('',*,*,#14014,.T.);
#18704=ORIENTED_EDGE('',*,*,#14015,.F.);
#18705=ORIENTED_EDGE('',*,*,#14016,.T.);
#18706=ORIENTED_EDGE('',*,*,#14017,.T.);
#18707=ORIENTED_EDGE('',*,*,#14018,.T.);
#18708=ORIENTED_EDGE('',*,*,#14019,.T.);
#18709=ORIENTED_EDGE('',*,*,#14020,.F.);
#18710=ORIENTED_EDGE('',*,*,#14021,.T.);
#18711=ORIENTED_EDGE('',*,*,#14022,.T.);
#18712=ORIENTED_EDGE('',*,*,#14023,.T.);
#18713=ORIENTED_EDGE('',*,*,#14024,.T.);
#18714=ORIENTED_EDGE('',*,*,#14017,.F.);
#18715=ORIENTED_EDGE('',*,*,#14025,.T.);
#18716=ORIENTED_EDGE('',*,*,#14026,.T.);
#18717=ORIENTED_EDGE('',*,*,#14027,.T.);
#18718=ORIENTED_EDGE('',*,*,#14028,.T.);
#18719=ORIENTED_EDGE('',*,*,#14023,.F.);
#18720=ORIENTED_EDGE('',*,*,#14029,.T.);
#18721=ORIENTED_EDGE('',*,*,#14030,.T.);
#18722=ORIENTED_EDGE('',*,*,#14031,.T.);
#18723=ORIENTED_EDGE('',*,*,#14032,.T.);
#18724=ORIENTED_EDGE('',*,*,#14033,.T.);
#18725=ORIENTED_EDGE('',*,*,#14026,.F.);
#18726=ORIENTED_EDGE('',*,*,#14034,.T.);
#18727=ORIENTED_EDGE('',*,*,#14035,.T.);
#18728=ORIENTED_EDGE('',*,*,#14036,.T.);
#18729=ORIENTED_EDGE('',*,*,#14037,.T.);
#18730=ORIENTED_EDGE('',*,*,#14031,.F.);
#18731=ORIENTED_EDGE('',*,*,#14038,.T.);
#18732=ORIENTED_EDGE('',*,*,#14039,.T.);
#18733=ORIENTED_EDGE('',*,*,#14040,.T.);
#18734=ORIENTED_EDGE('',*,*,#14041,.T.);
#18735=ORIENTED_EDGE('',*,*,#14035,.F.);
#18736=ORIENTED_EDGE('',*,*,#14042,.T.);
#18737=ORIENTED_EDGE('',*,*,#14043,.T.);
#18738=ORIENTED_EDGE('',*,*,#14044,.T.);
#18739=ORIENTED_EDGE('',*,*,#14045,.T.);
#18740=ORIENTED_EDGE('',*,*,#14040,.F.);
#18741=ORIENTED_EDGE('',*,*,#14046,.T.);
#18742=ORIENTED_EDGE('',*,*,#14047,.T.);
#18743=ORIENTED_EDGE('',*,*,#14048,.T.);
#18744=ORIENTED_EDGE('',*,*,#14049,.T.);
#18745=ORIENTED_EDGE('',*,*,#14043,.F.);
#18746=ORIENTED_EDGE('',*,*,#14050,.T.);
#18747=ORIENTED_EDGE('',*,*,#14051,.T.);
#18748=ORIENTED_EDGE('',*,*,#14052,.T.);
#18749=ORIENTED_EDGE('',*,*,#14053,.T.);
#18750=ORIENTED_EDGE('',*,*,#14048,.F.);
#18751=ORIENTED_EDGE('',*,*,#14054,.T.);
#18752=ORIENTED_EDGE('',*,*,#14055,.T.);
#18753=ORIENTED_EDGE('',*,*,#14056,.T.);
#18754=ORIENTED_EDGE('',*,*,#14057,.T.);
#18755=ORIENTED_EDGE('',*,*,#14058,.T.);
#18756=ORIENTED_EDGE('',*,*,#14051,.F.);
#18757=ORIENTED_EDGE('',*,*,#14059,.T.);
#18758=ORIENTED_EDGE('',*,*,#14060,.T.);
#18759=ORIENTED_EDGE('',*,*,#14061,.T.);
#18760=ORIENTED_EDGE('',*,*,#14062,.T.);
#18761=ORIENTED_EDGE('',*,*,#14056,.F.);
#18762=ORIENTED_EDGE('',*,*,#14063,.T.);
#18763=ORIENTED_EDGE('',*,*,#14064,.T.);
#18764=ORIENTED_EDGE('',*,*,#14065,.T.);
#18765=ORIENTED_EDGE('',*,*,#14066,.T.);
#18766=ORIENTED_EDGE('',*,*,#14060,.F.);
#18767=ORIENTED_EDGE('',*,*,#14067,.T.);
#18768=ORIENTED_EDGE('',*,*,#14068,.T.);
#18769=ORIENTED_EDGE('',*,*,#14069,.T.);
#18770=ORIENTED_EDGE('',*,*,#14070,.T.);
#18771=ORIENTED_EDGE('',*,*,#14071,.T.);
#18772=ORIENTED_EDGE('',*,*,#14065,.F.);
#18773=ORIENTED_EDGE('',*,*,#14072,.T.);
#18774=ORIENTED_EDGE('',*,*,#14073,.T.);
#18775=ORIENTED_EDGE('',*,*,#14074,.T.);
#18776=ORIENTED_EDGE('',*,*,#14075,.T.);
#18777=ORIENTED_EDGE('',*,*,#14069,.F.);
#18778=ORIENTED_EDGE('',*,*,#14076,.T.);
#18779=ORIENTED_EDGE('',*,*,#14077,.T.);
#18780=ORIENTED_EDGE('',*,*,#14078,.T.);
#18781=ORIENTED_EDGE('',*,*,#14079,.T.);
#18782=ORIENTED_EDGE('',*,*,#14074,.F.);
#18783=ORIENTED_EDGE('',*,*,#14080,.T.);
#18784=ORIENTED_EDGE('',*,*,#14081,.T.);
#18785=ORIENTED_EDGE('',*,*,#14082,.T.);
#18786=ORIENTED_EDGE('',*,*,#14083,.T.);
#18787=ORIENTED_EDGE('',*,*,#14084,.T.);
#18788=ORIENTED_EDGE('',*,*,#14077,.F.);
#18789=ORIENTED_EDGE('',*,*,#14085,.T.);
#18790=ORIENTED_EDGE('',*,*,#14086,.T.);
#18791=ORIENTED_EDGE('',*,*,#14087,.T.);
#18792=ORIENTED_EDGE('',*,*,#14088,.T.);
#18793=ORIENTED_EDGE('',*,*,#14082,.F.);
#18794=ORIENTED_EDGE('',*,*,#14089,.T.);
#18795=ORIENTED_EDGE('',*,*,#14090,.T.);
#18796=ORIENTED_EDGE('',*,*,#14091,.T.);
#18797=ORIENTED_EDGE('',*,*,#14092,.T.);
#18798=ORIENTED_EDGE('',*,*,#14086,.F.);
#18799=ORIENTED_EDGE('',*,*,#14093,.T.);
#18800=ORIENTED_EDGE('',*,*,#14094,.T.);
#18801=ORIENTED_EDGE('',*,*,#14095,.T.);
#18802=ORIENTED_EDGE('',*,*,#14096,.T.);
#18803=ORIENTED_EDGE('',*,*,#14097,.T.);
#18804=ORIENTED_EDGE('',*,*,#14091,.F.);
#18805=ORIENTED_EDGE('',*,*,#14098,.T.);
#18806=ORIENTED_EDGE('',*,*,#14099,.T.);
#18807=ORIENTED_EDGE('',*,*,#14100,.T.);
#18808=ORIENTED_EDGE('',*,*,#14101,.T.);
#18809=ORIENTED_EDGE('',*,*,#14095,.F.);
#18810=ORIENTED_EDGE('',*,*,#14102,.T.);
#18811=ORIENTED_EDGE('',*,*,#14103,.T.);
#18812=ORIENTED_EDGE('',*,*,#14104,.T.);
#18813=ORIENTED_EDGE('',*,*,#14105,.T.);
#18814=ORIENTED_EDGE('',*,*,#14100,.F.);
#18815=ORIENTED_EDGE('',*,*,#14106,.T.);
#18816=ORIENTED_EDGE('',*,*,#14107,.T.);
#18817=ORIENTED_EDGE('',*,*,#14108,.T.);
#18818=ORIENTED_EDGE('',*,*,#14109,.T.);
#18819=ORIENTED_EDGE('',*,*,#14103,.F.);
#18820=ORIENTED_EDGE('',*,*,#14110,.T.);
#18821=ORIENTED_EDGE('',*,*,#14111,.T.);
#18822=ORIENTED_EDGE('',*,*,#14112,.T.);
#18823=ORIENTED_EDGE('',*,*,#14113,.T.);
#18824=ORIENTED_EDGE('',*,*,#14108,.F.);
#18825=ORIENTED_EDGE('',*,*,#14114,.T.);
#18826=ORIENTED_EDGE('',*,*,#14115,.T.);
#18827=ORIENTED_EDGE('',*,*,#14116,.T.);
#18828=ORIENTED_EDGE('',*,*,#14117,.T.);
#18829=ORIENTED_EDGE('',*,*,#14111,.F.);
#18830=ORIENTED_EDGE('',*,*,#14118,.T.);
#18831=ORIENTED_EDGE('',*,*,#14119,.T.);
#18832=ORIENTED_EDGE('',*,*,#14120,.T.);
#18833=ORIENTED_EDGE('',*,*,#14121,.T.);
#18834=ORIENTED_EDGE('',*,*,#14122,.T.);
#18835=ORIENTED_EDGE('',*,*,#14116,.F.);
#18836=ORIENTED_EDGE('',*,*,#14123,.T.);
#18837=ORIENTED_EDGE('',*,*,#14124,.T.);
#18838=ORIENTED_EDGE('',*,*,#14125,.T.);
#18839=ORIENTED_EDGE('',*,*,#14126,.T.);
#18840=ORIENTED_EDGE('',*,*,#14120,.F.);
#18841=ORIENTED_EDGE('',*,*,#14127,.T.);
#18842=ORIENTED_EDGE('',*,*,#14128,.F.);
#18843=ORIENTED_EDGE('',*,*,#14129,.T.);
#18844=ORIENTED_EDGE('',*,*,#14130,.F.);
#18845=ORIENTED_EDGE('',*,*,#14131,.T.);
#18846=ORIENTED_EDGE('',*,*,#14132,.T.);
#18847=ORIENTED_EDGE('',*,*,#14133,.T.);
#18848=ORIENTED_EDGE('',*,*,#14134,.T.);
#18849=ORIENTED_EDGE('',*,*,#14135,.F.);
#18850=ORIENTED_EDGE('',*,*,#14136,.T.);
#18851=ORIENTED_EDGE('',*,*,#14137,.T.);
#18852=ORIENTED_EDGE('',*,*,#14138,.T.);
#18853=ORIENTED_EDGE('',*,*,#14139,.T.);
#18854=ORIENTED_EDGE('',*,*,#14132,.F.);
#18855=ORIENTED_EDGE('',*,*,#14140,.T.);
#18856=ORIENTED_EDGE('',*,*,#14141,.T.);
#18857=ORIENTED_EDGE('',*,*,#14142,.T.);
#18858=ORIENTED_EDGE('',*,*,#14143,.T.);
#18859=ORIENTED_EDGE('',*,*,#14138,.F.);
#18860=ORIENTED_EDGE('',*,*,#14144,.T.);
#18861=ORIENTED_EDGE('',*,*,#14145,.T.);
#18862=ORIENTED_EDGE('',*,*,#14146,.T.);
#18863=ORIENTED_EDGE('',*,*,#14147,.T.);
#18864=ORIENTED_EDGE('',*,*,#14148,.T.);
#18865=ORIENTED_EDGE('',*,*,#14141,.F.);
#18866=ORIENTED_EDGE('',*,*,#14149,.T.);
#18867=ORIENTED_EDGE('',*,*,#14150,.T.);
#18868=ORIENTED_EDGE('',*,*,#14151,.T.);
#18869=ORIENTED_EDGE('',*,*,#14152,.T.);
#18870=ORIENTED_EDGE('',*,*,#14146,.F.);
#18871=ORIENTED_EDGE('',*,*,#14153,.T.);
#18872=ORIENTED_EDGE('',*,*,#14154,.T.);
#18873=ORIENTED_EDGE('',*,*,#14155,.T.);
#18874=ORIENTED_EDGE('',*,*,#14156,.T.);
#18875=ORIENTED_EDGE('',*,*,#14150,.F.);
#18876=ORIENTED_EDGE('',*,*,#14157,.T.);
#18877=ORIENTED_EDGE('',*,*,#14158,.T.);
#18878=ORIENTED_EDGE('',*,*,#14159,.T.);
#18879=ORIENTED_EDGE('',*,*,#14160,.T.);
#18880=ORIENTED_EDGE('',*,*,#14155,.F.);
#18881=ORIENTED_EDGE('',*,*,#14161,.T.);
#18882=ORIENTED_EDGE('',*,*,#14162,.T.);
#18883=ORIENTED_EDGE('',*,*,#14163,.T.);
#18884=ORIENTED_EDGE('',*,*,#14164,.T.);
#18885=ORIENTED_EDGE('',*,*,#14158,.F.);
#18886=ORIENTED_EDGE('',*,*,#14165,.T.);
#18887=ORIENTED_EDGE('',*,*,#14166,.T.);
#18888=ORIENTED_EDGE('',*,*,#14167,.T.);
#18889=ORIENTED_EDGE('',*,*,#14168,.T.);
#18890=ORIENTED_EDGE('',*,*,#14163,.F.);
#18891=ORIENTED_EDGE('',*,*,#14169,.T.);
#18892=ORIENTED_EDGE('',*,*,#14170,.T.);
#18893=ORIENTED_EDGE('',*,*,#14171,.T.);
#18894=ORIENTED_EDGE('',*,*,#14172,.T.);
#18895=ORIENTED_EDGE('',*,*,#14173,.T.);
#18896=ORIENTED_EDGE('',*,*,#14166,.F.);
#18897=ORIENTED_EDGE('',*,*,#14174,.T.);
#18898=ORIENTED_EDGE('',*,*,#14175,.T.);
#18899=ORIENTED_EDGE('',*,*,#14176,.T.);
#18900=ORIENTED_EDGE('',*,*,#14177,.T.);
#18901=ORIENTED_EDGE('',*,*,#14171,.F.);
#18902=ORIENTED_EDGE('',*,*,#14178,.T.);
#18903=ORIENTED_EDGE('',*,*,#14179,.T.);
#18904=ORIENTED_EDGE('',*,*,#14180,.T.);
#18905=ORIENTED_EDGE('',*,*,#14181,.T.);
#18906=ORIENTED_EDGE('',*,*,#14175,.F.);
#18907=ORIENTED_EDGE('',*,*,#14182,.T.);
#18908=ORIENTED_EDGE('',*,*,#14183,.T.);
#18909=ORIENTED_EDGE('',*,*,#14184,.T.);
#18910=ORIENTED_EDGE('',*,*,#14185,.T.);
#18911=ORIENTED_EDGE('',*,*,#14186,.T.);
#18912=ORIENTED_EDGE('',*,*,#14180,.F.);
#18913=ORIENTED_EDGE('',*,*,#14187,.T.);
#18914=ORIENTED_EDGE('',*,*,#14188,.T.);
#18915=ORIENTED_EDGE('',*,*,#14189,.T.);
#18916=ORIENTED_EDGE('',*,*,#14190,.T.);
#18917=ORIENTED_EDGE('',*,*,#14184,.F.);
#18918=ORIENTED_EDGE('',*,*,#14191,.T.);
#18919=ORIENTED_EDGE('',*,*,#14192,.T.);
#18920=ORIENTED_EDGE('',*,*,#14193,.T.);
#18921=ORIENTED_EDGE('',*,*,#14194,.T.);
#18922=ORIENTED_EDGE('',*,*,#14189,.F.);
#18923=ORIENTED_EDGE('',*,*,#14195,.T.);
#18924=ORIENTED_EDGE('',*,*,#14196,.T.);
#18925=ORIENTED_EDGE('',*,*,#14197,.T.);
#18926=ORIENTED_EDGE('',*,*,#14198,.T.);
#18927=ORIENTED_EDGE('',*,*,#14199,.T.);
#18928=ORIENTED_EDGE('',*,*,#14192,.F.);
#18929=ORIENTED_EDGE('',*,*,#14200,.T.);
#18930=ORIENTED_EDGE('',*,*,#14201,.T.);
#18931=ORIENTED_EDGE('',*,*,#14202,.T.);
#18932=ORIENTED_EDGE('',*,*,#14203,.T.);
#18933=ORIENTED_EDGE('',*,*,#14197,.F.);
#18934=ORIENTED_EDGE('',*,*,#14204,.T.);
#18935=ORIENTED_EDGE('',*,*,#14205,.T.);
#18936=ORIENTED_EDGE('',*,*,#14206,.T.);
#18937=ORIENTED_EDGE('',*,*,#14207,.T.);
#18938=ORIENTED_EDGE('',*,*,#14201,.F.);
#18939=ORIENTED_EDGE('',*,*,#14208,.T.);
#18940=ORIENTED_EDGE('',*,*,#14209,.T.);
#18941=ORIENTED_EDGE('',*,*,#14210,.T.);
#18942=ORIENTED_EDGE('',*,*,#14211,.T.);
#18943=ORIENTED_EDGE('',*,*,#14212,.T.);
#18944=ORIENTED_EDGE('',*,*,#14206,.F.);
#18945=ORIENTED_EDGE('',*,*,#14213,.T.);
#18946=ORIENTED_EDGE('',*,*,#14214,.T.);
#18947=ORIENTED_EDGE('',*,*,#14215,.T.);
#18948=ORIENTED_EDGE('',*,*,#14216,.T.);
#18949=ORIENTED_EDGE('',*,*,#14210,.F.);
#18950=ORIENTED_EDGE('',*,*,#14217,.T.);
#18951=ORIENTED_EDGE('',*,*,#14218,.T.);
#18952=ORIENTED_EDGE('',*,*,#14219,.T.);
#18953=ORIENTED_EDGE('',*,*,#14220,.T.);
#18954=ORIENTED_EDGE('',*,*,#14215,.F.);
#18955=ORIENTED_EDGE('',*,*,#14221,.T.);
#18956=ORIENTED_EDGE('',*,*,#14222,.T.);
#18957=ORIENTED_EDGE('',*,*,#14223,.T.);
#18958=ORIENTED_EDGE('',*,*,#14224,.T.);
#18959=ORIENTED_EDGE('',*,*,#14218,.F.);
#18960=ORIENTED_EDGE('',*,*,#14225,.T.);
#18961=ORIENTED_EDGE('',*,*,#14226,.T.);
#18962=ORIENTED_EDGE('',*,*,#14227,.T.);
#18963=ORIENTED_EDGE('',*,*,#14228,.T.);
#18964=ORIENTED_EDGE('',*,*,#14223,.F.);
#18965=ORIENTED_EDGE('',*,*,#14229,.T.);
#18966=ORIENTED_EDGE('',*,*,#14230,.T.);
#18967=ORIENTED_EDGE('',*,*,#14231,.T.);
#18968=ORIENTED_EDGE('',*,*,#14232,.T.);
#18969=ORIENTED_EDGE('',*,*,#14226,.F.);
#18970=ORIENTED_EDGE('',*,*,#14233,.T.);
#18971=ORIENTED_EDGE('',*,*,#14234,.T.);
#18972=ORIENTED_EDGE('',*,*,#14235,.T.);
#18973=ORIENTED_EDGE('',*,*,#14236,.T.);
#18974=ORIENTED_EDGE('',*,*,#14237,.T.);
#18975=ORIENTED_EDGE('',*,*,#14231,.F.);
#18976=ORIENTED_EDGE('',*,*,#14238,.T.);
#18977=ORIENTED_EDGE('',*,*,#14239,.T.);
#18978=ORIENTED_EDGE('',*,*,#14240,.T.);
#18979=ORIENTED_EDGE('',*,*,#14241,.T.);
#18980=ORIENTED_EDGE('',*,*,#14235,.F.);
#18981=ORIENTED_EDGE('',*,*,#14242,.T.);
#18982=ORIENTED_EDGE('',*,*,#14243,.F.);
#18983=ORIENTED_EDGE('',*,*,#14244,.T.);
#18984=ORIENTED_EDGE('',*,*,#14245,.F.);
#18985=ORIENTED_EDGE('',*,*,#14246,.T.);
#18986=ORIENTED_EDGE('',*,*,#14247,.T.);
#18987=ORIENTED_EDGE('',*,*,#14248,.T.);
#18988=ORIENTED_EDGE('',*,*,#14249,.T.);
#18989=ORIENTED_EDGE('',*,*,#14250,.F.);
#18990=ORIENTED_EDGE('',*,*,#14251,.T.);
#18991=ORIENTED_EDGE('',*,*,#14252,.T.);
#18992=ORIENTED_EDGE('',*,*,#14253,.T.);
#18993=ORIENTED_EDGE('',*,*,#14254,.T.);
#18994=ORIENTED_EDGE('',*,*,#14247,.F.);
#18995=ORIENTED_EDGE('',*,*,#14255,.T.);
#18996=ORIENTED_EDGE('',*,*,#14256,.T.);
#18997=ORIENTED_EDGE('',*,*,#14257,.T.);
#18998=ORIENTED_EDGE('',*,*,#14258,.T.);
#18999=ORIENTED_EDGE('',*,*,#14253,.F.);
#19000=ORIENTED_EDGE('',*,*,#14259,.T.);
#19001=ORIENTED_EDGE('',*,*,#14260,.T.);
#19002=ORIENTED_EDGE('',*,*,#14261,.T.);
#19003=ORIENTED_EDGE('',*,*,#14262,.T.);
#19004=ORIENTED_EDGE('',*,*,#14263,.T.);
#19005=ORIENTED_EDGE('',*,*,#14256,.F.);
#19006=ORIENTED_EDGE('',*,*,#14264,.T.);
#19007=ORIENTED_EDGE('',*,*,#14265,.T.);
#19008=ORIENTED_EDGE('',*,*,#14266,.T.);
#19009=ORIENTED_EDGE('',*,*,#14267,.T.);
#19010=ORIENTED_EDGE('',*,*,#14261,.F.);
#19011=ORIENTED_EDGE('',*,*,#14268,.T.);
#19012=ORIENTED_EDGE('',*,*,#14269,.T.);
#19013=ORIENTED_EDGE('',*,*,#14270,.T.);
#19014=ORIENTED_EDGE('',*,*,#14271,.T.);
#19015=ORIENTED_EDGE('',*,*,#14265,.F.);
#19016=ORIENTED_EDGE('',*,*,#14272,.T.);
#19017=ORIENTED_EDGE('',*,*,#14273,.T.);
#19018=ORIENTED_EDGE('',*,*,#14274,.T.);
#19019=ORIENTED_EDGE('',*,*,#14275,.T.);
#19020=ORIENTED_EDGE('',*,*,#14270,.F.);
#19021=ORIENTED_EDGE('',*,*,#14276,.T.);
#19022=ORIENTED_EDGE('',*,*,#14277,.T.);
#19023=ORIENTED_EDGE('',*,*,#14278,.T.);
#19024=ORIENTED_EDGE('',*,*,#14279,.T.);
#19025=ORIENTED_EDGE('',*,*,#14273,.F.);
#19026=ORIENTED_EDGE('',*,*,#14280,.T.);
#19027=ORIENTED_EDGE('',*,*,#14281,.T.);
#19028=ORIENTED_EDGE('',*,*,#14282,.T.);
#19029=ORIENTED_EDGE('',*,*,#14283,.T.);
#19030=ORIENTED_EDGE('',*,*,#14278,.F.);
#19031=ORIENTED_EDGE('',*,*,#14284,.T.);
#19032=ORIENTED_EDGE('',*,*,#14285,.T.);
#19033=ORIENTED_EDGE('',*,*,#14286,.T.);
#19034=ORIENTED_EDGE('',*,*,#14287,.T.);
#19035=ORIENTED_EDGE('',*,*,#14288,.T.);
#19036=ORIENTED_EDGE('',*,*,#14281,.F.);
#19037=ORIENTED_EDGE('',*,*,#14289,.T.);
#19038=ORIENTED_EDGE('',*,*,#14290,.T.);
#19039=ORIENTED_EDGE('',*,*,#14291,.T.);
#19040=ORIENTED_EDGE('',*,*,#14292,.T.);
#19041=ORIENTED_EDGE('',*,*,#14286,.F.);
#19042=ORIENTED_EDGE('',*,*,#14293,.T.);
#19043=ORIENTED_EDGE('',*,*,#14294,.T.);
#19044=ORIENTED_EDGE('',*,*,#14295,.T.);
#19045=ORIENTED_EDGE('',*,*,#14296,.T.);
#19046=ORIENTED_EDGE('',*,*,#14290,.F.);
#19047=ORIENTED_EDGE('',*,*,#14297,.T.);
#19048=ORIENTED_EDGE('',*,*,#14298,.T.);
#19049=ORIENTED_EDGE('',*,*,#14299,.T.);
#19050=ORIENTED_EDGE('',*,*,#14300,.T.);
#19051=ORIENTED_EDGE('',*,*,#14301,.T.);
#19052=ORIENTED_EDGE('',*,*,#14295,.F.);
#19053=ORIENTED_EDGE('',*,*,#14302,.T.);
#19054=ORIENTED_EDGE('',*,*,#14303,.T.);
#19055=ORIENTED_EDGE('',*,*,#14304,.T.);
#19056=ORIENTED_EDGE('',*,*,#14305,.T.);
#19057=ORIENTED_EDGE('',*,*,#14299,.F.);
#19058=ORIENTED_EDGE('',*,*,#14306,.T.);
#19059=ORIENTED_EDGE('',*,*,#14307,.T.);
#19060=ORIENTED_EDGE('',*,*,#14308,.T.);
#19061=ORIENTED_EDGE('',*,*,#14309,.T.);
#19062=ORIENTED_EDGE('',*,*,#14304,.F.);
#19063=ORIENTED_EDGE('',*,*,#14310,.T.);
#19064=ORIENTED_EDGE('',*,*,#14311,.T.);
#19065=ORIENTED_EDGE('',*,*,#14312,.T.);
#19066=ORIENTED_EDGE('',*,*,#14313,.T.);
#19067=ORIENTED_EDGE('',*,*,#14314,.T.);
#19068=ORIENTED_EDGE('',*,*,#14307,.F.);
#19069=ORIENTED_EDGE('',*,*,#14315,.T.);
#19070=ORIENTED_EDGE('',*,*,#14316,.T.);
#19071=ORIENTED_EDGE('',*,*,#14317,.T.);
#19072=ORIENTED_EDGE('',*,*,#14318,.T.);
#19073=ORIENTED_EDGE('',*,*,#14312,.F.);
#19074=ORIENTED_EDGE('',*,*,#14319,.T.);
#19075=ORIENTED_EDGE('',*,*,#14320,.T.);
#19076=ORIENTED_EDGE('',*,*,#14321,.T.);
#19077=ORIENTED_EDGE('',*,*,#14322,.T.);
#19078=ORIENTED_EDGE('',*,*,#14316,.F.);
#19079=ORIENTED_EDGE('',*,*,#14323,.T.);
#19080=ORIENTED_EDGE('',*,*,#14324,.T.);
#19081=ORIENTED_EDGE('',*,*,#14325,.T.);
#19082=ORIENTED_EDGE('',*,*,#14326,.T.);
#19083=ORIENTED_EDGE('',*,*,#14327,.T.);
#19084=ORIENTED_EDGE('',*,*,#14321,.F.);
#19085=ORIENTED_EDGE('',*,*,#14328,.T.);
#19086=ORIENTED_EDGE('',*,*,#14329,.T.);
#19087=ORIENTED_EDGE('',*,*,#14330,.T.);
#19088=ORIENTED_EDGE('',*,*,#14331,.T.);
#19089=ORIENTED_EDGE('',*,*,#14325,.F.);
#19090=ORIENTED_EDGE('',*,*,#14332,.T.);
#19091=ORIENTED_EDGE('',*,*,#14333,.T.);
#19092=ORIENTED_EDGE('',*,*,#14334,.T.);
#19093=ORIENTED_EDGE('',*,*,#14335,.T.);
#19094=ORIENTED_EDGE('',*,*,#14330,.F.);
#19095=ORIENTED_EDGE('',*,*,#14336,.T.);
#19096=ORIENTED_EDGE('',*,*,#14337,.T.);
#19097=ORIENTED_EDGE('',*,*,#14338,.T.);
#19098=ORIENTED_EDGE('',*,*,#14339,.T.);
#19099=ORIENTED_EDGE('',*,*,#14333,.F.);
#19100=ORIENTED_EDGE('',*,*,#14340,.T.);
#19101=ORIENTED_EDGE('',*,*,#14341,.T.);
#19102=ORIENTED_EDGE('',*,*,#14342,.T.);
#19103=ORIENTED_EDGE('',*,*,#14343,.T.);
#19104=ORIENTED_EDGE('',*,*,#14338,.F.);
#19105=ORIENTED_EDGE('',*,*,#14344,.T.);
#19106=ORIENTED_EDGE('',*,*,#14345,.T.);
#19107=ORIENTED_EDGE('',*,*,#14346,.T.);
#19108=ORIENTED_EDGE('',*,*,#14347,.T.);
#19109=ORIENTED_EDGE('',*,*,#14341,.F.);
#19110=ORIENTED_EDGE('',*,*,#14348,.T.);
#19111=ORIENTED_EDGE('',*,*,#14349,.T.);
#19112=ORIENTED_EDGE('',*,*,#14350,.T.);
#19113=ORIENTED_EDGE('',*,*,#14351,.T.);
#19114=ORIENTED_EDGE('',*,*,#14352,.T.);
#19115=ORIENTED_EDGE('',*,*,#14346,.F.);
#19116=ORIENTED_EDGE('',*,*,#14353,.T.);
#19117=ORIENTED_EDGE('',*,*,#14354,.T.);
#19118=ORIENTED_EDGE('',*,*,#14355,.T.);
#19119=ORIENTED_EDGE('',*,*,#14356,.T.);
#19120=ORIENTED_EDGE('',*,*,#14350,.F.);
#19121=ORIENTED_EDGE('',*,*,#14357,.T.);
#19122=ORIENTED_EDGE('',*,*,#14358,.F.);
#19123=ORIENTED_EDGE('',*,*,#14359,.T.);
#19124=ORIENTED_EDGE('',*,*,#14360,.F.);
#19125=ORIENTED_EDGE('',*,*,#14361,.T.);
#19126=ORIENTED_EDGE('',*,*,#14358,.T.);
#19127=ORIENTED_EDGE('',*,*,#14362,.T.);
#19128=ORIENTED_EDGE('',*,*,#14363,.T.);
#19129=ORIENTED_EDGE('',*,*,#14355,.F.);
#19130=ORIENTED_EDGE('',*,*,#14364,.T.);
#19131=ORIENTED_EDGE('',*,*,#14365,.T.);
#19132=ORIENTED_EDGE('',*,*,#14243,.T.);
#19133=ORIENTED_EDGE('',*,*,#14366,.T.);
#19134=ORIENTED_EDGE('',*,*,#14367,.T.);
#19135=ORIENTED_EDGE('',*,*,#14240,.F.);
#19136=ORIENTED_EDGE('',*,*,#14368,.T.);
#19137=ORIENTED_EDGE('',*,*,#14369,.T.);
#19138=ORIENTED_EDGE('',*,*,#14128,.T.);
#19139=ORIENTED_EDGE('',*,*,#14370,.T.);
#19140=ORIENTED_EDGE('',*,*,#14371,.T.);
#19141=ORIENTED_EDGE('',*,*,#14125,.F.);
#19142=ORIENTED_EDGE('',*,*,#14372,.T.);
#19143=ORIENTED_EDGE('',*,*,#14373,.T.);
#19144=ORIENTED_EDGE('',*,*,#14013,.T.);
#19145=ORIENTED_EDGE('',*,*,#14374,.T.);
#19146=ORIENTED_EDGE('',*,*,#14375,.T.);
#19147=ORIENTED_EDGE('',*,*,#14010,.F.);
#19148=ORIENTED_EDGE('',*,*,#14376,.T.);
#19149=ORIENTED_EDGE('',*,*,#14377,.T.);
#19150=ORIENTED_EDGE('',*,*,#13897,.T.);
#19151=ORIENTED_EDGE('',*,*,#14378,.T.);
#19152=ORIENTED_EDGE('',*,*,#14379,.T.);
#19153=ORIENTED_EDGE('',*,*,#13892,.F.);
#19154=ORIENTED_EDGE('',*,*,#14380,.T.);
#19155=ORIENTED_EDGE('',*,*,#14381,.T.);
#19156=ORIENTED_EDGE('',*,*,#13882,.T.);
#19157=ORIENTED_EDGE('',*,*,#14382,.T.);
#19158=ORIENTED_EDGE('',*,*,#13877,.F.);
#19159=ORIENTED_EDGE('',*,*,#14383,.T.);
#19160=ORIENTED_EDGE('',*,*,#14384,.F.);
#19161=ORIENTED_EDGE('',*,*,#13861,.T.);
#19162=ORIENTED_EDGE('',*,*,#14385,.T.);
#19163=ORIENTED_EDGE('',*,*,#14386,.T.);
#19164=ORIENTED_EDGE('',*,*,#13856,.F.);
#19165=ORIENTED_EDGE('',*,*,#14387,.F.);
#19166=ORIENTED_EDGE('',*,*,#14388,.F.);
#19167=ORIENTED_EDGE('',*,*,#13724,.T.);
#19168=ORIENTED_EDGE('',*,*,#14389,.T.);
#19169=ORIENTED_EDGE('',*,*,#14390,.T.);
#19170=ORIENTED_EDGE('',*,*,#13719,.F.);
#19171=ORIENTED_EDGE('',*,*,#14391,.F.);
#19172=ORIENTED_EDGE('',*,*,#14392,.F.);
#19173=ORIENTED_EDGE('',*,*,#13587,.T.);
#19174=ORIENTED_EDGE('',*,*,#14393,.T.);
#19175=ORIENTED_EDGE('',*,*,#14394,.T.);
#19176=ORIENTED_EDGE('',*,*,#13582,.F.);
#19177=ORIENTED_EDGE('',*,*,#14395,.F.);
#19178=ORIENTED_EDGE('',*,*,#14396,.F.);
#19179=ORIENTED_EDGE('',*,*,#13450,.T.);
#19180=ORIENTED_EDGE('',*,*,#14397,.T.);
#19181=ORIENTED_EDGE('',*,*,#14398,.T.);
#19182=ORIENTED_EDGE('',*,*,#13445,.F.);
#19183=ORIENTED_EDGE('',*,*,#14399,.F.);
#19184=ORIENTED_EDGE('',*,*,#14400,.F.);
#19185=ORIENTED_EDGE('',*,*,#13313,.T.);
#19186=ORIENTED_EDGE('',*,*,#14401,.T.);
#19187=ORIENTED_EDGE('',*,*,#14402,.T.);
#19188=ORIENTED_EDGE('',*,*,#13308,.F.);
#19189=ORIENTED_EDGE('',*,*,#14403,.F.);
#19190=ORIENTED_EDGE('',*,*,#14404,.F.);
#19191=ORIENTED_EDGE('',*,*,#13293,.T.);
#19192=ORIENTED_EDGE('',*,*,#14405,.T.);
#19193=ORIENTED_EDGE('',*,*,#14406,.T.);
#19194=ORIENTED_EDGE('',*,*,#13288,.F.);
#19195=ORIENTED_EDGE('',*,*,#14407,.F.);
#19196=ORIENTED_EDGE('',*,*,#14408,.F.);
#19197=ORIENTED_EDGE('',*,*,#14409,.F.);
#19198=ORIENTED_EDGE('',*,*,#14410,.T.);
#19199=ORIENTED_EDGE('',*,*,#14411,.T.);
#19200=ORIENTED_EDGE('',*,*,#14410,.F.);
#19201=ORIENTED_EDGE('',*,*,#14411,.F.);
#19202=ORIENTED_EDGE('',*,*,#14412,.F.);
#19203=ORIENTED_EDGE('',*,*,#14413,.F.);
#19204=ORIENTED_EDGE('',*,*,#14414,.T.);
#19205=ORIENTED_EDGE('',*,*,#14415,.F.);
#19206=ORIENTED_EDGE('',*,*,#14416,.F.);
#19207=ORIENTED_EDGE('',*,*,#14414,.F.);
#19208=ORIENTED_EDGE('',*,*,#14417,.F.);
#19209=ORIENTED_EDGE('',*,*,#14418,.F.);
#19210=ORIENTED_EDGE('',*,*,#14419,.F.);
#19211=ORIENTED_EDGE('',*,*,#14420,.F.);
#19212=ORIENTED_EDGE('',*,*,#14421,.T.);
#19213=ORIENTED_EDGE('',*,*,#14422,.T.);
#19214=ORIENTED_EDGE('',*,*,#14421,.F.);
#19215=ORIENTED_EDGE('',*,*,#14422,.F.);
#19216=ORIENTED_EDGE('',*,*,#14423,.F.);
#19217=ORIENTED_EDGE('',*,*,#14424,.F.);
#19218=ORIENTED_EDGE('',*,*,#14425,.T.);
#19219=ORIENTED_EDGE('',*,*,#14426,.F.);
#19220=ORIENTED_EDGE('',*,*,#14427,.F.);
#19221=ORIENTED_EDGE('',*,*,#14428,.F.);
#19222=ORIENTED_EDGE('',*,*,#14425,.F.);
#19223=ORIENTED_EDGE('',*,*,#14429,.F.);
#19224=ORIENTED_EDGE('',*,*,#14430,.F.);
#19225=ORIENTED_EDGE('',*,*,#14431,.F.);
#19226=ORIENTED_EDGE('',*,*,#14432,.T.);
#19227=ORIENTED_EDGE('',*,*,#14433,.T.);
#19228=ORIENTED_EDGE('',*,*,#14432,.F.);
#19229=ORIENTED_EDGE('',*,*,#14433,.F.);
#19230=ORIENTED_EDGE('',*,*,#14418,.T.);
#19231=ORIENTED_EDGE('',*,*,#14434,.F.);
#19232=ORIENTED_EDGE('',*,*,#14435,.T.);
#19233=ORIENTED_EDGE('',*,*,#14436,.T.);
#19234=ORIENTED_EDGE('',*,*,#14429,.T.);
#19235=ORIENTED_EDGE('',*,*,#14424,.T.);
#19236=ORIENTED_EDGE('',*,*,#14437,.F.);
#19237=ORIENTED_EDGE('',*,*,#14438,.F.);
#19238=ORIENTED_EDGE('',*,*,#14439,.F.);
#19239=ORIENTED_EDGE('',*,*,#14440,.T.);
#19240=ORIENTED_EDGE('',*,*,#14417,.T.);
#19241=ORIENTED_EDGE('',*,*,#14413,.T.);
#19242=ORIENTED_EDGE('',*,*,#14441,.F.);
#19243=ORIENTED_EDGE('',*,*,#14426,.T.);
#19244=ORIENTED_EDGE('',*,*,#14428,.T.);
#19245=ORIENTED_EDGE('',*,*,#14442,.F.);
#19246=ORIENTED_EDGE('',*,*,#14443,.F.);
#19247=ORIENTED_EDGE('',*,*,#14434,.T.);
#19248=ORIENTED_EDGE('',*,*,#14412,.T.);
#19249=ORIENTED_EDGE('',*,*,#14444,.T.);
#19250=ORIENTED_EDGE('',*,*,#14445,.T.);
#19251=ORIENTED_EDGE('',*,*,#14446,.T.);
#19252=ORIENTED_EDGE('',*,*,#14447,.T.);
#19253=ORIENTED_EDGE('',*,*,#14448,.T.);
#19254=ORIENTED_EDGE('',*,*,#14449,.T.);
#19255=ORIENTED_EDGE('',*,*,#14450,.T.);
#19256=ORIENTED_EDGE('',*,*,#14451,.T.);
#19257=ORIENTED_EDGE('',*,*,#14452,.T.);
#19258=ORIENTED_EDGE('',*,*,#14453,.T.);
#19259=ORIENTED_EDGE('',*,*,#14454,.T.);
#19260=ORIENTED_EDGE('',*,*,#14455,.T.);
#19261=ORIENTED_EDGE('',*,*,#14456,.T.);
#19262=ORIENTED_EDGE('',*,*,#14457,.T.);
#19263=ORIENTED_EDGE('',*,*,#14458,.T.);
#19264=ORIENTED_EDGE('',*,*,#14459,.T.);
#19265=ORIENTED_EDGE('',*,*,#14460,.T.);
#19266=ORIENTED_EDGE('',*,*,#14461,.T.);
#19267=ORIENTED_EDGE('',*,*,#14462,.T.);
#19268=ORIENTED_EDGE('',*,*,#14463,.T.);
#19269=ORIENTED_EDGE('',*,*,#14464,.T.);
#19270=ORIENTED_EDGE('',*,*,#14465,.T.);
#19271=ORIENTED_EDGE('',*,*,#14466,.T.);
#19272=ORIENTED_EDGE('',*,*,#14467,.T.);
#19273=ORIENTED_EDGE('',*,*,#14468,.T.);
#19274=ORIENTED_EDGE('',*,*,#14469,.T.);
#19275=ORIENTED_EDGE('',*,*,#14470,.T.);
#19276=ORIENTED_EDGE('',*,*,#14471,.T.);
#19277=ORIENTED_EDGE('',*,*,#14437,.T.);
#19278=ORIENTED_EDGE('',*,*,#14423,.T.);
#19279=ORIENTED_EDGE('',*,*,#14441,.T.);
#19280=ORIENTED_EDGE('',*,*,#14472,.T.);
#19281=ORIENTED_EDGE('',*,*,#14473,.T.);
#19282=ORIENTED_EDGE('',*,*,#14474,.T.);
#19283=ORIENTED_EDGE('',*,*,#13322,.T.);
#19284=ORIENTED_EDGE('',*,*,#14475,.T.);
#19285=ORIENTED_EDGE('',*,*,#14250,.T.);
#19286=ORIENTED_EDGE('',*,*,#14476,.T.);
#19287=ORIENTED_EDGE('',*,*,#13459,.T.);
#19288=ORIENTED_EDGE('',*,*,#14477,.T.);
#19289=ORIENTED_EDGE('',*,*,#14135,.T.);
#19290=ORIENTED_EDGE('',*,*,#14478,.T.);
#19291=ORIENTED_EDGE('',*,*,#13596,.T.);
#19292=ORIENTED_EDGE('',*,*,#14479,.T.);
#19293=ORIENTED_EDGE('',*,*,#14020,.T.);
#19294=ORIENTED_EDGE('',*,*,#14480,.T.);
#19295=ORIENTED_EDGE('',*,*,#13733,.T.);
#19296=ORIENTED_EDGE('',*,*,#14481,.T.);
#19297=ORIENTED_EDGE('',*,*,#13905,.T.);
#19298=ORIENTED_EDGE('',*,*,#14431,.T.);
#19299=ORIENTED_EDGE('',*,*,#14420,.T.);
#19300=ORIENTED_EDGE('',*,*,#14409,.T.);
#19301=ORIENTED_EDGE('',*,*,#14482,.F.);
#19302=ORIENTED_EDGE('',*,*,#13280,.F.);
#19303=ORIENTED_EDGE('',*,*,#13285,.F.);
#19304=ORIENTED_EDGE('',*,*,#13284,.F.);
#19305=ORIENTED_EDGE('',*,*,#13290,.F.);
#19306=ORIENTED_EDGE('',*,*,#13289,.F.);
#19307=ORIENTED_EDGE('',*,*,#14406,.F.);
#19308=ORIENTED_EDGE('',*,*,#14405,.F.);
#19309=ORIENTED_EDGE('',*,*,#13298,.F.);
#19310=ORIENTED_EDGE('',*,*,#13297,.F.);
#19311=ORIENTED_EDGE('',*,*,#14483,.F.);
#19312=ORIENTED_EDGE('',*,*,#13898,.F.);
#19313=ORIENTED_EDGE('',*,*,#14381,.F.);
#19314=ORIENTED_EDGE('',*,*,#14380,.F.);
#19315=ORIENTED_EDGE('',*,*,#13896,.F.);
#19316=ORIENTED_EDGE('',*,*,#13895,.F.);
#19317=ORIENTED_EDGE('',*,*,#13891,.F.);
#19318=ORIENTED_EDGE('',*,*,#13887,.F.);
#19319=ORIENTED_EDGE('',*,*,#14484,.F.);
#19320=ORIENTED_EDGE('',*,*,#13889,.F.);
#19321=ORIENTED_EDGE('',*,*,#13894,.F.);
#19322=ORIENTED_EDGE('',*,*,#13893,.F.);
#19323=ORIENTED_EDGE('',*,*,#14379,.F.);
#19324=ORIENTED_EDGE('',*,*,#14378,.F.);
#19325=ORIENTED_EDGE('',*,*,#13901,.F.);
#19326=ORIENTED_EDGE('',*,*,#13900,.F.);
#19327=ORIENTED_EDGE('',*,*,#14485,.F.);
#19328=ORIENTED_EDGE('',*,*,#13295,.T.);
#19329=ORIENTED_EDGE('',*,*,#13294,.T.);
#19330=ORIENTED_EDGE('',*,*,#14408,.T.);
#19331=ORIENTED_EDGE('',*,*,#14407,.T.);
#19332=ORIENTED_EDGE('',*,*,#13292,.T.);
#19333=ORIENTED_EDGE('',*,*,#13291,.T.);
#19334=ORIENTED_EDGE('',*,*,#13287,.T.);
#19335=ORIENTED_EDGE('',*,*,#13286,.T.);
#19336=ORIENTED_EDGE('',*,*,#13282,.T.);
#19337=ORIENTED_EDGE('',*,*,#14486,.F.);
#19338=ORIENTED_EDGE('',*,*,#13300,.F.);
#19339=ORIENTED_EDGE('',*,*,#13305,.F.);
#19340=ORIENTED_EDGE('',*,*,#13304,.F.);
#19341=ORIENTED_EDGE('',*,*,#13310,.F.);
#19342=ORIENTED_EDGE('',*,*,#13309,.F.);
#19343=ORIENTED_EDGE('',*,*,#14402,.F.);
#19344=ORIENTED_EDGE('',*,*,#14401,.F.);
#19345=ORIENTED_EDGE('',*,*,#13318,.F.);
#19346=ORIENTED_EDGE('',*,*,#13317,.F.);
#19347=ORIENTED_EDGE('',*,*,#14487,.F.);
#19348=ORIENTED_EDGE('',*,*,#13868,.F.);
#19349=ORIENTED_EDGE('',*,*,#13874,.F.);
#19350=ORIENTED_EDGE('',*,*,#13873,.F.);
#19351=ORIENTED_EDGE('',*,*,#13879,.F.);
#19352=ORIENTED_EDGE('',*,*,#13878,.F.);
#19353=ORIENTED_EDGE('',*,*,#14382,.F.);
#19354=ORIENTED_EDGE('',*,*,#13884,.F.);
#19355=ORIENTED_EDGE('',*,*,#14488,.F.);
#19356=ORIENTED_EDGE('',*,*,#14383,.F.);
#19357=ORIENTED_EDGE('',*,*,#13881,.F.);
#19358=ORIENTED_EDGE('',*,*,#13880,.F.);
#19359=ORIENTED_EDGE('',*,*,#13876,.F.);
#19360=ORIENTED_EDGE('',*,*,#13875,.F.);
#19361=ORIENTED_EDGE('',*,*,#13871,.F.);
#19362=ORIENTED_EDGE('',*,*,#13870,.F.);
#19363=ORIENTED_EDGE('',*,*,#14489,.F.);
#19364=ORIENTED_EDGE('',*,*,#13315,.T.);
#19365=ORIENTED_EDGE('',*,*,#13314,.T.);
#19366=ORIENTED_EDGE('',*,*,#14404,.T.);
#19367=ORIENTED_EDGE('',*,*,#14403,.T.);
#19368=ORIENTED_EDGE('',*,*,#13312,.T.);
#19369=ORIENTED_EDGE('',*,*,#13311,.T.);
#19370=ORIENTED_EDGE('',*,*,#13307,.T.);
#19371=ORIENTED_EDGE('',*,*,#13306,.T.);
#19372=ORIENTED_EDGE('',*,*,#13302,.T.);
#19373=ORIENTED_EDGE('',*,*,#14475,.F.);
#19374=ORIENTED_EDGE('',*,*,#13321,.F.);
#19375=ORIENTED_EDGE('',*,*,#13320,.F.);
#19376=ORIENTED_EDGE('',*,*,#13327,.F.);
#19377=ORIENTED_EDGE('',*,*,#13326,.F.);
#19378=ORIENTED_EDGE('',*,*,#13332,.F.);
#19379=ORIENTED_EDGE('',*,*,#13331,.F.);
#19380=ORIENTED_EDGE('',*,*,#13337,.F.);
#19381=ORIENTED_EDGE('',*,*,#13336,.F.);
#19382=ORIENTED_EDGE('',*,*,#13342,.F.);
#19383=ORIENTED_EDGE('',*,*,#13341,.F.);
#19384=ORIENTED_EDGE('',*,*,#13347,.F.);
#19385=ORIENTED_EDGE('',*,*,#13346,.F.);
#19386=ORIENTED_EDGE('',*,*,#13352,.F.);
#19387=ORIENTED_EDGE('',*,*,#13351,.F.);
#19388=ORIENTED_EDGE('',*,*,#13357,.F.);
#19389=ORIENTED_EDGE('',*,*,#13356,.F.);
#19390=ORIENTED_EDGE('',*,*,#13362,.F.);
#19391=ORIENTED_EDGE('',*,*,#13361,.F.);
#19392=ORIENTED_EDGE('',*,*,#13367,.F.);
#19393=ORIENTED_EDGE('',*,*,#13366,.F.);
#19394=ORIENTED_EDGE('',*,*,#13372,.F.);
#19395=ORIENTED_EDGE('',*,*,#13371,.F.);
#19396=ORIENTED_EDGE('',*,*,#13377,.F.);
#19397=ORIENTED_EDGE('',*,*,#13376,.F.);
#19398=ORIENTED_EDGE('',*,*,#13382,.F.);
#19399=ORIENTED_EDGE('',*,*,#13381,.F.);
#19400=ORIENTED_EDGE('',*,*,#13387,.F.);
#19401=ORIENTED_EDGE('',*,*,#13386,.F.);
#19402=ORIENTED_EDGE('',*,*,#13392,.F.);
#19403=ORIENTED_EDGE('',*,*,#13391,.F.);
#19404=ORIENTED_EDGE('',*,*,#13397,.F.);
#19405=ORIENTED_EDGE('',*,*,#13396,.F.);
#19406=ORIENTED_EDGE('',*,*,#13402,.F.);
#19407=ORIENTED_EDGE('',*,*,#13401,.F.);
#19408=ORIENTED_EDGE('',*,*,#13407,.F.);
#19409=ORIENTED_EDGE('',*,*,#13406,.F.);
#19410=ORIENTED_EDGE('',*,*,#13412,.F.);
#19411=ORIENTED_EDGE('',*,*,#13411,.F.);
#19412=ORIENTED_EDGE('',*,*,#13417,.F.);
#19413=ORIENTED_EDGE('',*,*,#13416,.F.);
#19414=ORIENTED_EDGE('',*,*,#13422,.F.);
#19415=ORIENTED_EDGE('',*,*,#13421,.F.);
#19416=ORIENTED_EDGE('',*,*,#13427,.F.);
#19417=ORIENTED_EDGE('',*,*,#13426,.F.);
#19418=ORIENTED_EDGE('',*,*,#13432,.F.);
#19419=ORIENTED_EDGE('',*,*,#13431,.F.);
#19420=ORIENTED_EDGE('',*,*,#13437,.F.);
#19421=ORIENTED_EDGE('',*,*,#13436,.F.);
#19422=ORIENTED_EDGE('',*,*,#13442,.F.);
#19423=ORIENTED_EDGE('',*,*,#13441,.F.);
#19424=ORIENTED_EDGE('',*,*,#13447,.F.);
#19425=ORIENTED_EDGE('',*,*,#13446,.F.);
#19426=ORIENTED_EDGE('',*,*,#14398,.F.);
#19427=ORIENTED_EDGE('',*,*,#14397,.F.);
#19428=ORIENTED_EDGE('',*,*,#13455,.F.);
#19429=ORIENTED_EDGE('',*,*,#13454,.F.);
#19430=ORIENTED_EDGE('',*,*,#14490,.F.);
#19431=ORIENTED_EDGE('',*,*,#14359,.F.);
#19432=ORIENTED_EDGE('',*,*,#14365,.F.);
#19433=ORIENTED_EDGE('',*,*,#14364,.F.);
#19434=ORIENTED_EDGE('',*,*,#14357,.F.);
#19435=ORIENTED_EDGE('',*,*,#14354,.F.);
#19436=ORIENTED_EDGE('',*,*,#14353,.F.);
#19437=ORIENTED_EDGE('',*,*,#14349,.F.);
#19438=ORIENTED_EDGE('',*,*,#14348,.F.);
#19439=ORIENTED_EDGE('',*,*,#14345,.F.);
#19440=ORIENTED_EDGE('',*,*,#14344,.F.);
#19441=ORIENTED_EDGE('',*,*,#14340,.F.);
#19442=ORIENTED_EDGE('',*,*,#14337,.F.);
#19443=ORIENTED_EDGE('',*,*,#14336,.F.);
#19444=ORIENTED_EDGE('',*,*,#14332,.F.);
#19445=ORIENTED_EDGE('',*,*,#14329,.F.);
#19446=ORIENTED_EDGE('',*,*,#14328,.F.);
#19447=ORIENTED_EDGE('',*,*,#14324,.F.);
#19448=ORIENTED_EDGE('',*,*,#14323,.F.);
#19449=ORIENTED_EDGE('',*,*,#14320,.F.);
#19450=ORIENTED_EDGE('',*,*,#14319,.F.);
#19451=ORIENTED_EDGE('',*,*,#14315,.F.);
#19452=ORIENTED_EDGE('',*,*,#14311,.F.);
#19453=ORIENTED_EDGE('',*,*,#14310,.F.);
#19454=ORIENTED_EDGE('',*,*,#14306,.F.);
#19455=ORIENTED_EDGE('',*,*,#14303,.F.);
#19456=ORIENTED_EDGE('',*,*,#14302,.F.);
#19457=ORIENTED_EDGE('',*,*,#14298,.F.);
#19458=ORIENTED_EDGE('',*,*,#14297,.F.);
#19459=ORIENTED_EDGE('',*,*,#14294,.F.);
#19460=ORIENTED_EDGE('',*,*,#14293,.F.);
#19461=ORIENTED_EDGE('',*,*,#14289,.F.);
#19462=ORIENTED_EDGE('',*,*,#14285,.F.);
#19463=ORIENTED_EDGE('',*,*,#14284,.F.);
#19464=ORIENTED_EDGE('',*,*,#14280,.F.);
#19465=ORIENTED_EDGE('',*,*,#14277,.F.);
#19466=ORIENTED_EDGE('',*,*,#14276,.F.);
#19467=ORIENTED_EDGE('',*,*,#14272,.F.);
#19468=ORIENTED_EDGE('',*,*,#14269,.F.);
#19469=ORIENTED_EDGE('',*,*,#14268,.F.);
#19470=ORIENTED_EDGE('',*,*,#14264,.F.);
#19471=ORIENTED_EDGE('',*,*,#14260,.F.);
#19472=ORIENTED_EDGE('',*,*,#14259,.F.);
#19473=ORIENTED_EDGE('',*,*,#14255,.F.);
#19474=ORIENTED_EDGE('',*,*,#14252,.F.);
#19475=ORIENTED_EDGE('',*,*,#14251,.F.);
#19476=ORIENTED_EDGE('',*,*,#14474,.F.);
#19477=ORIENTED_EDGE('',*,*,#14249,.F.);
#19478=ORIENTED_EDGE('',*,*,#14248,.F.);
#19479=ORIENTED_EDGE('',*,*,#14254,.F.);
#19480=ORIENTED_EDGE('',*,*,#14258,.F.);
#19481=ORIENTED_EDGE('',*,*,#14257,.F.);
#19482=ORIENTED_EDGE('',*,*,#14263,.F.);
#19483=ORIENTED_EDGE('',*,*,#14262,.F.);
#19484=ORIENTED_EDGE('',*,*,#14267,.F.);
#19485=ORIENTED_EDGE('',*,*,#14266,.F.);
#19486=ORIENTED_EDGE('',*,*,#14271,.F.);
#19487=ORIENTED_EDGE('',*,*,#14275,.F.);
#19488=ORIENTED_EDGE('',*,*,#14274,.F.);
#19489=ORIENTED_EDGE('',*,*,#14279,.F.);
#19490=ORIENTED_EDGE('',*,*,#14283,.F.);
#19491=ORIENTED_EDGE('',*,*,#14282,.F.);
#19492=ORIENTED_EDGE('',*,*,#14288,.F.);
#19493=ORIENTED_EDGE('',*,*,#14287,.F.);
#19494=ORIENTED_EDGE('',*,*,#14292,.F.);
#19495=ORIENTED_EDGE('',*,*,#14291,.F.);
#19496=ORIENTED_EDGE('',*,*,#14296,.F.);
#19497=ORIENTED_EDGE('',*,*,#14301,.F.);
#19498=ORIENTED_EDGE('',*,*,#14300,.F.);
#19499=ORIENTED_EDGE('',*,*,#14305,.F.);
#19500=ORIENTED_EDGE('',*,*,#14309,.F.);
#19501=ORIENTED_EDGE('',*,*,#14308,.F.);
#19502=ORIENTED_EDGE('',*,*,#14314,.F.);
#19503=ORIENTED_EDGE('',*,*,#14313,.F.);
#19504=ORIENTED_EDGE('',*,*,#14318,.F.);
#19505=ORIENTED_EDGE('',*,*,#14317,.F.);
#19506=ORIENTED_EDGE('',*,*,#14322,.F.);
#19507=ORIENTED_EDGE('',*,*,#14327,.F.);
#19508=ORIENTED_EDGE('',*,*,#14326,.F.);
#19509=ORIENTED_EDGE('',*,*,#14331,.F.);
#19510=ORIENTED_EDGE('',*,*,#14335,.F.);
#19511=ORIENTED_EDGE('',*,*,#14334,.F.);
#19512=ORIENTED_EDGE('',*,*,#14339,.F.);
#19513=ORIENTED_EDGE('',*,*,#14343,.F.);
#19514=ORIENTED_EDGE('',*,*,#14342,.F.);
#19515=ORIENTED_EDGE('',*,*,#14347,.F.);
#19516=ORIENTED_EDGE('',*,*,#14352,.F.);
#19517=ORIENTED_EDGE('',*,*,#14351,.F.);
#19518=ORIENTED_EDGE('',*,*,#14356,.F.);
#19519=ORIENTED_EDGE('',*,*,#14363,.F.);
#19520=ORIENTED_EDGE('',*,*,#14362,.F.);
#19521=ORIENTED_EDGE('',*,*,#14361,.F.);
#19522=ORIENTED_EDGE('',*,*,#14491,.F.);
#19523=ORIENTED_EDGE('',*,*,#13452,.T.);
#19524=ORIENTED_EDGE('',*,*,#13451,.T.);
#19525=ORIENTED_EDGE('',*,*,#14400,.T.);
#19526=ORIENTED_EDGE('',*,*,#14399,.T.);
#19527=ORIENTED_EDGE('',*,*,#13449,.T.);
#19528=ORIENTED_EDGE('',*,*,#13448,.T.);
#19529=ORIENTED_EDGE('',*,*,#13444,.T.);
#19530=ORIENTED_EDGE('',*,*,#13443,.T.);
#19531=ORIENTED_EDGE('',*,*,#13439,.T.);
#19532=ORIENTED_EDGE('',*,*,#13438,.T.);
#19533=ORIENTED_EDGE('',*,*,#13434,.T.);
#19534=ORIENTED_EDGE('',*,*,#13433,.T.);
#19535=ORIENTED_EDGE('',*,*,#13429,.T.);
#19536=ORIENTED_EDGE('',*,*,#13428,.T.);
#19537=ORIENTED_EDGE('',*,*,#13424,.T.);
#19538=ORIENTED_EDGE('',*,*,#13423,.T.);
#19539=ORIENTED_EDGE('',*,*,#13419,.T.);
#19540=ORIENTED_EDGE('',*,*,#13418,.T.);
#19541=ORIENTED_EDGE('',*,*,#13414,.T.);
#19542=ORIENTED_EDGE('',*,*,#13413,.T.);
#19543=ORIENTED_EDGE('',*,*,#13409,.T.);
#19544=ORIENTED_EDGE('',*,*,#13408,.T.);
#19545=ORIENTED_EDGE('',*,*,#13404,.T.);
#19546=ORIENTED_EDGE('',*,*,#13403,.T.);
#19547=ORIENTED_EDGE('',*,*,#13399,.T.);
#19548=ORIENTED_EDGE('',*,*,#13398,.T.);
#19549=ORIENTED_EDGE('',*,*,#13394,.T.);
#19550=ORIENTED_EDGE('',*,*,#13393,.T.);
#19551=ORIENTED_EDGE('',*,*,#13389,.T.);
#19552=ORIENTED_EDGE('',*,*,#13388,.T.);
#19553=ORIENTED_EDGE('',*,*,#13384,.T.);
#19554=ORIENTED_EDGE('',*,*,#13383,.T.);
#19555=ORIENTED_EDGE('',*,*,#13379,.T.);
#19556=ORIENTED_EDGE('',*,*,#13378,.T.);
#19557=ORIENTED_EDGE('',*,*,#13374,.T.);
#19558=ORIENTED_EDGE('',*,*,#13373,.T.);
#19559=ORIENTED_EDGE('',*,*,#13369,.T.);
#19560=ORIENTED_EDGE('',*,*,#13368,.T.);
#19561=ORIENTED_EDGE('',*,*,#13364,.T.);
#19562=ORIENTED_EDGE('',*,*,#13363,.T.);
#19563=ORIENTED_EDGE('',*,*,#13359,.T.);
#19564=ORIENTED_EDGE('',*,*,#13358,.T.);
#19565=ORIENTED_EDGE('',*,*,#13354,.T.);
#19566=ORIENTED_EDGE('',*,*,#13353,.T.);
#19567=ORIENTED_EDGE('',*,*,#13349,.T.);
#19568=ORIENTED_EDGE('',*,*,#13348,.T.);
#19569=ORIENTED_EDGE('',*,*,#13344,.T.);
#19570=ORIENTED_EDGE('',*,*,#13343,.T.);
#19571=ORIENTED_EDGE('',*,*,#13339,.T.);
#19572=ORIENTED_EDGE('',*,*,#13338,.T.);
#19573=ORIENTED_EDGE('',*,*,#13334,.T.);
#19574=ORIENTED_EDGE('',*,*,#13333,.T.);
#19575=ORIENTED_EDGE('',*,*,#13329,.T.);
#19576=ORIENTED_EDGE('',*,*,#13328,.T.);
#19577=ORIENTED_EDGE('',*,*,#13324,.T.);
#19578=ORIENTED_EDGE('',*,*,#13323,.T.);
#19579=ORIENTED_EDGE('',*,*,#14477,.F.);
#19580=ORIENTED_EDGE('',*,*,#13458,.F.);
#19581=ORIENTED_EDGE('',*,*,#13457,.F.);
#19582=ORIENTED_EDGE('',*,*,#13464,.F.);
#19583=ORIENTED_EDGE('',*,*,#13463,.F.);
#19584=ORIENTED_EDGE('',*,*,#13469,.F.);
#19585=ORIENTED_EDGE('',*,*,#13468,.F.);
#19586=ORIENTED_EDGE('',*,*,#13474,.F.);
#19587=ORIENTED_EDGE('',*,*,#13473,.F.);
#19588=ORIENTED_EDGE('',*,*,#13479,.F.);
#19589=ORIENTED_EDGE('',*,*,#13478,.F.);
#19590=ORIENTED_EDGE('',*,*,#13484,.F.);
#19591=ORIENTED_EDGE('',*,*,#13483,.F.);
#19592=ORIENTED_EDGE('',*,*,#13489,.F.);
#19593=ORIENTED_EDGE('',*,*,#13488,.F.);
#19594=ORIENTED_EDGE('',*,*,#13494,.F.);
#19595=ORIENTED_EDGE('',*,*,#13493,.F.);
#19596=ORIENTED_EDGE('',*,*,#13499,.F.);
#19597=ORIENTED_EDGE('',*,*,#13498,.F.);
#19598=ORIENTED_EDGE('',*,*,#13504,.F.);
#19599=ORIENTED_EDGE('',*,*,#13503,.F.);
#19600=ORIENTED_EDGE('',*,*,#13509,.F.);
#19601=ORIENTED_EDGE('',*,*,#13508,.F.);
#19602=ORIENTED_EDGE('',*,*,#13514,.F.);
#19603=ORIENTED_EDGE('',*,*,#13513,.F.);
#19604=ORIENTED_EDGE('',*,*,#13519,.F.);
#19605=ORIENTED_EDGE('',*,*,#13518,.F.);
#19606=ORIENTED_EDGE('',*,*,#13524,.F.);
#19607=ORIENTED_EDGE('',*,*,#13523,.F.);
#19608=ORIENTED_EDGE('',*,*,#13529,.F.);
#19609=ORIENTED_EDGE('',*,*,#13528,.F.);
#19610=ORIENTED_EDGE('',*,*,#13534,.F.);
#19611=ORIENTED_EDGE('',*,*,#13533,.F.);
#19612=ORIENTED_EDGE('',*,*,#13539,.F.);
#19613=ORIENTED_EDGE('',*,*,#13538,.F.);
#19614=ORIENTED_EDGE('',*,*,#13544,.F.);
#19615=ORIENTED_EDGE('',*,*,#13543,.F.);
#19616=ORIENTED_EDGE('',*,*,#13549,.F.);
#19617=ORIENTED_EDGE('',*,*,#13548,.F.);
#19618=ORIENTED_EDGE('',*,*,#13554,.F.);
#19619=ORIENTED_EDGE('',*,*,#13553,.F.);
#19620=ORIENTED_EDGE('',*,*,#13559,.F.);
#19621=ORIENTED_EDGE('',*,*,#13558,.F.);
#19622=ORIENTED_EDGE('',*,*,#13564,.F.);
#19623=ORIENTED_EDGE('',*,*,#13563,.F.);
#19624=ORIENTED_EDGE('',*,*,#13569,.F.);
#19625=ORIENTED_EDGE('',*,*,#13568,.F.);
#19626=ORIENTED_EDGE('',*,*,#13574,.F.);
#19627=ORIENTED_EDGE('',*,*,#13573,.F.);
#19628=ORIENTED_EDGE('',*,*,#13579,.F.);
#19629=ORIENTED_EDGE('',*,*,#13578,.F.);
#19630=ORIENTED_EDGE('',*,*,#13584,.F.);
#19631=ORIENTED_EDGE('',*,*,#13583,.F.);
#19632=ORIENTED_EDGE('',*,*,#14394,.F.);
#19633=ORIENTED_EDGE('',*,*,#14393,.F.);
#19634=ORIENTED_EDGE('',*,*,#13592,.F.);
#19635=ORIENTED_EDGE('',*,*,#13591,.F.);
#19636=ORIENTED_EDGE('',*,*,#14492,.F.);
#19637=ORIENTED_EDGE('',*,*,#14244,.F.);
#19638=ORIENTED_EDGE('',*,*,#14369,.F.);
#19639=ORIENTED_EDGE('',*,*,#14368,.F.);
#19640=ORIENTED_EDGE('',*,*,#14242,.F.);
#19641=ORIENTED_EDGE('',*,*,#14239,.F.);
#19642=ORIENTED_EDGE('',*,*,#14238,.F.);
#19643=ORIENTED_EDGE('',*,*,#14234,.F.);
#19644=ORIENTED_EDGE('',*,*,#14233,.F.);
#19645=ORIENTED_EDGE('',*,*,#14230,.F.);
#19646=ORIENTED_EDGE('',*,*,#14229,.F.);
#19647=ORIENTED_EDGE('',*,*,#14225,.F.);
#19648=ORIENTED_EDGE('',*,*,#14222,.F.);
#19649=ORIENTED_EDGE('',*,*,#14221,.F.);
#19650=ORIENTED_EDGE('',*,*,#14217,.F.);
#19651=ORIENTED_EDGE('',*,*,#14214,.F.);
#19652=ORIENTED_EDGE('',*,*,#14213,.F.);
#19653=ORIENTED_EDGE('',*,*,#14209,.F.);
#19654=ORIENTED_EDGE('',*,*,#14208,.F.);
#19655=ORIENTED_EDGE('',*,*,#14205,.F.);
#19656=ORIENTED_EDGE('',*,*,#14204,.F.);
#19657=ORIENTED_EDGE('',*,*,#14200,.F.);
#19658=ORIENTED_EDGE('',*,*,#14196,.F.);
#19659=ORIENTED_EDGE('',*,*,#14195,.F.);
#19660=ORIENTED_EDGE('',*,*,#14191,.F.);
#19661=ORIENTED_EDGE('',*,*,#14188,.F.);
#19662=ORIENTED_EDGE('',*,*,#14187,.F.);
#19663=ORIENTED_EDGE('',*,*,#14183,.F.);
#19664=ORIENTED_EDGE('',*,*,#14182,.F.);
#19665=ORIENTED_EDGE('',*,*,#14179,.F.);
#19666=ORIENTED_EDGE('',*,*,#14178,.F.);
#19667=ORIENTED_EDGE('',*,*,#14174,.F.);
#19668=ORIENTED_EDGE('',*,*,#14170,.F.);
#19669=ORIENTED_EDGE('',*,*,#14169,.F.);
#19670=ORIENTED_EDGE('',*,*,#14165,.F.);
#19671=ORIENTED_EDGE('',*,*,#14162,.F.);
#19672=ORIENTED_EDGE('',*,*,#14161,.F.);
#19673=ORIENTED_EDGE('',*,*,#14157,.F.);
#19674=ORIENTED_EDGE('',*,*,#14154,.F.);
#19675=ORIENTED_EDGE('',*,*,#14153,.F.);
#19676=ORIENTED_EDGE('',*,*,#14149,.F.);
#19677=ORIENTED_EDGE('',*,*,#14145,.F.);
#19678=ORIENTED_EDGE('',*,*,#14144,.F.);
#19679=ORIENTED_EDGE('',*,*,#14140,.F.);
#19680=ORIENTED_EDGE('',*,*,#14137,.F.);
#19681=ORIENTED_EDGE('',*,*,#14136,.F.);
#19682=ORIENTED_EDGE('',*,*,#14476,.F.);
#19683=ORIENTED_EDGE('',*,*,#14134,.F.);
#19684=ORIENTED_EDGE('',*,*,#14133,.F.);
#19685=ORIENTED_EDGE('',*,*,#14139,.F.);
#19686=ORIENTED_EDGE('',*,*,#14143,.F.);
#19687=ORIENTED_EDGE('',*,*,#14142,.F.);
#19688=ORIENTED_EDGE('',*,*,#14148,.F.);
#19689=ORIENTED_EDGE('',*,*,#14147,.F.);
#19690=ORIENTED_EDGE('',*,*,#14152,.F.);
#19691=ORIENTED_EDGE('',*,*,#14151,.F.);
#19692=ORIENTED_EDGE('',*,*,#14156,.F.);
#19693=ORIENTED_EDGE('',*,*,#14160,.F.);
#19694=ORIENTED_EDGE('',*,*,#14159,.F.);
#19695=ORIENTED_EDGE('',*,*,#14164,.F.);
#19696=ORIENTED_EDGE('',*,*,#14168,.F.);
#19697=ORIENTED_EDGE('',*,*,#14167,.F.);
#19698=ORIENTED_EDGE('',*,*,#14173,.F.);
#19699=ORIENTED_EDGE('',*,*,#14172,.F.);
#19700=ORIENTED_EDGE('',*,*,#14177,.F.);
#19701=ORIENTED_EDGE('',*,*,#14176,.F.);
#19702=ORIENTED_EDGE('',*,*,#14181,.F.);
#19703=ORIENTED_EDGE('',*,*,#14186,.F.);
#19704=ORIENTED_EDGE('',*,*,#14185,.F.);
#19705=ORIENTED_EDGE('',*,*,#14190,.F.);
#19706=ORIENTED_EDGE('',*,*,#14194,.F.);
#19707=ORIENTED_EDGE('',*,*,#14193,.F.);
#19708=ORIENTED_EDGE('',*,*,#14199,.F.);
#19709=ORIENTED_EDGE('',*,*,#14198,.F.);
#19710=ORIENTED_EDGE('',*,*,#14203,.F.);
#19711=ORIENTED_EDGE('',*,*,#14202,.F.);
#19712=ORIENTED_EDGE('',*,*,#14207,.F.);
#19713=ORIENTED_EDGE('',*,*,#14212,.F.);
#19714=ORIENTED_EDGE('',*,*,#14211,.F.);
#19715=ORIENTED_EDGE('',*,*,#14216,.F.);
#19716=ORIENTED_EDGE('',*,*,#14220,.F.);
#19717=ORIENTED_EDGE('',*,*,#14219,.F.);
#19718=ORIENTED_EDGE('',*,*,#14224,.F.);
#19719=ORIENTED_EDGE('',*,*,#14228,.F.);
#19720=ORIENTED_EDGE('',*,*,#14227,.F.);
#19721=ORIENTED_EDGE('',*,*,#14232,.F.);
#19722=ORIENTED_EDGE('',*,*,#14237,.F.);
#19723=ORIENTED_EDGE('',*,*,#14236,.F.);
#19724=ORIENTED_EDGE('',*,*,#14241,.F.);
#19725=ORIENTED_EDGE('',*,*,#14367,.F.);
#19726=ORIENTED_EDGE('',*,*,#14366,.F.);
#19727=ORIENTED_EDGE('',*,*,#14246,.F.);
#19728=ORIENTED_EDGE('',*,*,#14493,.F.);
#19729=ORIENTED_EDGE('',*,*,#13589,.T.);
#19730=ORIENTED_EDGE('',*,*,#13588,.T.);
#19731=ORIENTED_EDGE('',*,*,#14396,.T.);
#19732=ORIENTED_EDGE('',*,*,#14395,.T.);
#19733=ORIENTED_EDGE('',*,*,#13586,.T.);
#19734=ORIENTED_EDGE('',*,*,#13585,.T.);
#19735=ORIENTED_EDGE('',*,*,#13581,.T.);
#19736=ORIENTED_EDGE('',*,*,#13580,.T.);
#19737=ORIENTED_EDGE('',*,*,#13576,.T.);
#19738=ORIENTED_EDGE('',*,*,#13575,.T.);
#19739=ORIENTED_EDGE('',*,*,#13571,.T.);
#19740=ORIENTED_EDGE('',*,*,#13570,.T.);
#19741=ORIENTED_EDGE('',*,*,#13566,.T.);
#19742=ORIENTED_EDGE('',*,*,#13565,.T.);
#19743=ORIENTED_EDGE('',*,*,#13561,.T.);
#19744=ORIENTED_EDGE('',*,*,#13560,.T.);
#19745=ORIENTED_EDGE('',*,*,#13556,.T.);
#19746=ORIENTED_EDGE('',*,*,#13555,.T.);
#19747=ORIENTED_EDGE('',*,*,#13551,.T.);
#19748=ORIENTED_EDGE('',*,*,#13550,.T.);
#19749=ORIENTED_EDGE('',*,*,#13546,.T.);
#19750=ORIENTED_EDGE('',*,*,#13545,.T.);
#19751=ORIENTED_EDGE('',*,*,#13541,.T.);
#19752=ORIENTED_EDGE('',*,*,#13540,.T.);
#19753=ORIENTED_EDGE('',*,*,#13536,.T.);
#19754=ORIENTED_EDGE('',*,*,#13535,.T.);
#19755=ORIENTED_EDGE('',*,*,#13531,.T.);
#19756=ORIENTED_EDGE('',*,*,#13530,.T.);
#19757=ORIENTED_EDGE('',*,*,#13526,.T.);
#19758=ORIENTED_EDGE('',*,*,#13525,.T.);
#19759=ORIENTED_EDGE('',*,*,#13521,.T.);
#19760=ORIENTED_EDGE('',*,*,#13520,.T.);
#19761=ORIENTED_EDGE('',*,*,#13516,.T.);
#19762=ORIENTED_EDGE('',*,*,#13515,.T.);
#19763=ORIENTED_EDGE('',*,*,#13511,.T.);
#19764=ORIENTED_EDGE('',*,*,#13510,.T.);
#19765=ORIENTED_EDGE('',*,*,#13506,.T.);
#19766=ORIENTED_EDGE('',*,*,#13505,.T.);
#19767=ORIENTED_EDGE('',*,*,#13501,.T.);
#19768=ORIENTED_EDGE('',*,*,#13500,.T.);
#19769=ORIENTED_EDGE('',*,*,#13496,.T.);
#19770=ORIENTED_EDGE('',*,*,#13495,.T.);
#19771=ORIENTED_EDGE('',*,*,#13491,.T.);
#19772=ORIENTED_EDGE('',*,*,#13490,.T.);
#19773=ORIENTED_EDGE('',*,*,#13486,.T.);
#19774=ORIENTED_EDGE('',*,*,#13485,.T.);
#19775=ORIENTED_EDGE('',*,*,#13481,.T.);
#19776=ORIENTED_EDGE('',*,*,#13480,.T.);
#19777=ORIENTED_EDGE('',*,*,#13476,.T.);
#19778=ORIENTED_EDGE('',*,*,#13475,.T.);
#19779=ORIENTED_EDGE('',*,*,#13471,.T.);
#19780=ORIENTED_EDGE('',*,*,#13470,.T.);
#19781=ORIENTED_EDGE('',*,*,#13466,.T.);
#19782=ORIENTED_EDGE('',*,*,#13465,.T.);
#19783=ORIENTED_EDGE('',*,*,#13461,.T.);
#19784=ORIENTED_EDGE('',*,*,#13460,.T.);
#19785=ORIENTED_EDGE('',*,*,#14479,.F.);
#19786=ORIENTED_EDGE('',*,*,#13595,.F.);
#19787=ORIENTED_EDGE('',*,*,#13594,.F.);
#19788=ORIENTED_EDGE('',*,*,#13601,.F.);
#19789=ORIENTED_EDGE('',*,*,#13600,.F.);
#19790=ORIENTED_EDGE('',*,*,#13606,.F.);
#19791=ORIENTED_EDGE('',*,*,#13605,.F.);
#19792=ORIENTED_EDGE('',*,*,#13611,.F.);
#19793=ORIENTED_EDGE('',*,*,#13610,.F.);
#19794=ORIENTED_EDGE('',*,*,#13616,.F.);
#19795=ORIENTED_EDGE('',*,*,#13615,.F.);
#19796=ORIENTED_EDGE('',*,*,#13621,.F.);
#19797=ORIENTED_EDGE('',*,*,#13620,.F.);
#19798=ORIENTED_EDGE('',*,*,#13626,.F.);
#19799=ORIENTED_EDGE('',*,*,#13625,.F.);
#19800=ORIENTED_EDGE('',*,*,#13631,.F.);
#19801=ORIENTED_EDGE('',*,*,#13630,.F.);
#19802=ORIENTED_EDGE('',*,*,#13636,.F.);
#19803=ORIENTED_EDGE('',*,*,#13635,.F.);
#19804=ORIENTED_EDGE('',*,*,#13641,.F.);
#19805=ORIENTED_EDGE('',*,*,#13640,.F.);
#19806=ORIENTED_EDGE('',*,*,#13646,.F.);
#19807=ORIENTED_EDGE('',*,*,#13645,.F.);
#19808=ORIENTED_EDGE('',*,*,#13651,.F.);
#19809=ORIENTED_EDGE('',*,*,#13650,.F.);
#19810=ORIENTED_EDGE('',*,*,#13656,.F.);
#19811=ORIENTED_EDGE('',*,*,#13655,.F.);
#19812=ORIENTED_EDGE('',*,*,#13661,.F.);
#19813=ORIENTED_EDGE('',*,*,#13660,.F.);
#19814=ORIENTED_EDGE('',*,*,#13666,.F.);
#19815=ORIENTED_EDGE('',*,*,#13665,.F.);
#19816=ORIENTED_EDGE('',*,*,#13671,.F.);
#19817=ORIENTED_EDGE('',*,*,#13670,.F.);
#19818=ORIENTED_EDGE('',*,*,#13676,.F.);
#19819=ORIENTED_EDGE('',*,*,#13675,.F.);
#19820=ORIENTED_EDGE('',*,*,#13681,.F.);
#19821=ORIENTED_EDGE('',*,*,#13680,.F.);
#19822=ORIENTED_EDGE('',*,*,#13686,.F.);
#19823=ORIENTED_EDGE('',*,*,#13685,.F.);
#19824=ORIENTED_EDGE('',*,*,#13691,.F.);
#19825=ORIENTED_EDGE('',*,*,#13690,.F.);
#19826=ORIENTED_EDGE('',*,*,#13696,.F.);
#19827=ORIENTED_EDGE('',*,*,#13695,.F.);
#19828=ORIENTED_EDGE('',*,*,#13701,.F.);
#19829=ORIENTED_EDGE('',*,*,#13700,.F.);
#19830=ORIENTED_EDGE('',*,*,#13706,.F.);
#19831=ORIENTED_EDGE('',*,*,#13705,.F.);
#19832=ORIENTED_EDGE('',*,*,#13711,.F.);
#19833=ORIENTED_EDGE('',*,*,#13710,.F.);
#19834=ORIENTED_EDGE('',*,*,#13716,.F.);
#19835=ORIENTED_EDGE('',*,*,#13715,.F.);
#19836=ORIENTED_EDGE('',*,*,#13721,.F.);
#19837=ORIENTED_EDGE('',*,*,#13720,.F.);
#19838=ORIENTED_EDGE('',*,*,#14390,.F.);
#19839=ORIENTED_EDGE('',*,*,#14389,.F.);
#19840=ORIENTED_EDGE('',*,*,#13729,.F.);
#19841=ORIENTED_EDGE('',*,*,#13728,.F.);
#19842=ORIENTED_EDGE('',*,*,#14494,.F.);
#19843=ORIENTED_EDGE('',*,*,#14129,.F.);
#19844=ORIENTED_EDGE('',*,*,#14373,.F.);
#19845=ORIENTED_EDGE('',*,*,#14372,.F.);
#19846=ORIENTED_EDGE('',*,*,#14127,.F.);
#19847=ORIENTED_EDGE('',*,*,#14124,.F.);
#19848=ORIENTED_EDGE('',*,*,#14123,.F.);
#19849=ORIENTED_EDGE('',*,*,#14119,.F.);
#19850=ORIENTED_EDGE('',*,*,#14118,.F.);
#19851=ORIENTED_EDGE('',*,*,#14115,.F.);
#19852=ORIENTED_EDGE('',*,*,#14114,.F.);
#19853=ORIENTED_EDGE('',*,*,#14110,.F.);
#19854=ORIENTED_EDGE('',*,*,#14107,.F.);
#19855=ORIENTED_EDGE('',*,*,#14106,.F.);
#19856=ORIENTED_EDGE('',*,*,#14102,.F.);
#19857=ORIENTED_EDGE('',*,*,#14099,.F.);
#19858=ORIENTED_EDGE('',*,*,#14098,.F.);
#19859=ORIENTED_EDGE('',*,*,#14094,.F.);
#19860=ORIENTED_EDGE('',*,*,#14093,.F.);
#19861=ORIENTED_EDGE('',*,*,#14090,.F.);
#19862=ORIENTED_EDGE('',*,*,#14089,.F.);
#19863=ORIENTED_EDGE('',*,*,#14085,.F.);
#19864=ORIENTED_EDGE('',*,*,#14081,.F.);
#19865=ORIENTED_EDGE('',*,*,#14080,.F.);
#19866=ORIENTED_EDGE('',*,*,#14076,.F.);
#19867=ORIENTED_EDGE('',*,*,#14073,.F.);
#19868=ORIENTED_EDGE('',*,*,#14072,.F.);
#19869=ORIENTED_EDGE('',*,*,#14068,.F.);
#19870=ORIENTED_EDGE('',*,*,#14067,.F.);
#19871=ORIENTED_EDGE('',*,*,#14064,.F.);
#19872=ORIENTED_EDGE('',*,*,#14063,.F.);
#19873=ORIENTED_EDGE('',*,*,#14059,.F.);
#19874=ORIENTED_EDGE('',*,*,#14055,.F.);
#19875=ORIENTED_EDGE('',*,*,#14054,.F.);
#19876=ORIENTED_EDGE('',*,*,#14050,.F.);
#19877=ORIENTED_EDGE('',*,*,#14047,.F.);
#19878=ORIENTED_EDGE('',*,*,#14046,.F.);
#19879=ORIENTED_EDGE('',*,*,#14042,.F.);
#19880=ORIENTED_EDGE('',*,*,#14039,.F.);
#19881=ORIENTED_EDGE('',*,*,#14038,.F.);
#19882=ORIENTED_EDGE('',*,*,#14034,.F.);
#19883=ORIENTED_EDGE('',*,*,#14030,.F.);
#19884=ORIENTED_EDGE('',*,*,#14029,.F.);
#19885=ORIENTED_EDGE('',*,*,#14025,.F.);
#19886=ORIENTED_EDGE('',*,*,#14022,.F.);
#19887=ORIENTED_EDGE('',*,*,#14021,.F.);
#19888=ORIENTED_EDGE('',*,*,#14478,.F.);
#19889=ORIENTED_EDGE('',*,*,#14019,.F.);
#19890=ORIENTED_EDGE('',*,*,#14018,.F.);
#19891=ORIENTED_EDGE('',*,*,#14024,.F.);
#19892=ORIENTED_EDGE('',*,*,#14028,.F.);
#19893=ORIENTED_EDGE('',*,*,#14027,.F.);
#19894=ORIENTED_EDGE('',*,*,#14033,.F.);
#19895=ORIENTED_EDGE('',*,*,#14032,.F.);
#19896=ORIENTED_EDGE('',*,*,#14037,.F.);
#19897=ORIENTED_EDGE('',*,*,#14036,.F.);
#19898=ORIENTED_EDGE('',*,*,#14041,.F.);
#19899=ORIENTED_EDGE('',*,*,#14045,.F.);
#19900=ORIENTED_EDGE('',*,*,#14044,.F.);
#19901=ORIENTED_EDGE('',*,*,#14049,.F.);
#19902=ORIENTED_EDGE('',*,*,#14053,.F.);
#19903=ORIENTED_EDGE('',*,*,#14052,.F.);
#19904=ORIENTED_EDGE('',*,*,#14058,.F.);
#19905=ORIENTED_EDGE('',*,*,#14057,.F.);
#19906=ORIENTED_EDGE('',*,*,#14062,.F.);
#19907=ORIENTED_EDGE('',*,*,#14061,.F.);
#19908=ORIENTED_EDGE('',*,*,#14066,.F.);
#19909=ORIENTED_EDGE('',*,*,#14071,.F.);
#19910=ORIENTED_EDGE('',*,*,#14070,.F.);
#19911=ORIENTED_EDGE('',*,*,#14075,.F.);
#19912=ORIENTED_EDGE('',*,*,#14079,.F.);
#19913=ORIENTED_EDGE('',*,*,#14078,.F.);
#19914=ORIENTED_EDGE('',*,*,#14084,.F.);
#19915=ORIENTED_EDGE('',*,*,#14083,.F.);
#19916=ORIENTED_EDGE('',*,*,#14088,.F.);
#19917=ORIENTED_EDGE('',*,*,#14087,.F.);
#19918=ORIENTED_EDGE('',*,*,#14092,.F.);
#19919=ORIENTED_EDGE('',*,*,#14097,.F.);
#19920=ORIENTED_EDGE('',*,*,#14096,.F.);
#19921=ORIENTED_EDGE('',*,*,#14101,.F.);
#19922=ORIENTED_EDGE('',*,*,#14105,.F.);
#19923=ORIENTED_EDGE('',*,*,#14104,.F.);
#19924=ORIENTED_EDGE('',*,*,#14109,.F.);
#19925=ORIENTED_EDGE('',*,*,#14113,.F.);
#19926=ORIENTED_EDGE('',*,*,#14112,.F.);
#19927=ORIENTED_EDGE('',*,*,#14117,.F.);
#19928=ORIENTED_EDGE('',*,*,#14122,.F.);
#19929=ORIENTED_EDGE('',*,*,#14121,.F.);
#19930=ORIENTED_EDGE('',*,*,#14126,.F.);
#19931=ORIENTED_EDGE('',*,*,#14371,.F.);
#19932=ORIENTED_EDGE('',*,*,#14370,.F.);
#19933=ORIENTED_EDGE('',*,*,#14131,.F.);
#19934=ORIENTED_EDGE('',*,*,#14495,.F.);
#19935=ORIENTED_EDGE('',*,*,#13726,.T.);
#19936=ORIENTED_EDGE('',*,*,#13725,.T.);
#19937=ORIENTED_EDGE('',*,*,#14392,.T.);
#19938=ORIENTED_EDGE('',*,*,#14391,.T.);
#19939=ORIENTED_EDGE('',*,*,#13723,.T.);
#19940=ORIENTED_EDGE('',*,*,#13722,.T.);
#19941=ORIENTED_EDGE('',*,*,#13718,.T.);
#19942=ORIENTED_EDGE('',*,*,#13717,.T.);
#19943=ORIENTED_EDGE('',*,*,#13713,.T.);
#19944=ORIENTED_EDGE('',*,*,#13712,.T.);
#19945=ORIENTED_EDGE('',*,*,#13708,.T.);
#19946=ORIENTED_EDGE('',*,*,#13707,.T.);
#19947=ORIENTED_EDGE('',*,*,#13703,.T.);
#19948=ORIENTED_EDGE('',*,*,#13702,.T.);
#19949=ORIENTED_EDGE('',*,*,#13698,.T.);
#19950=ORIENTED_EDGE('',*,*,#13697,.T.);
#19951=ORIENTED_EDGE('',*,*,#13693,.T.);
#19952=ORIENTED_EDGE('',*,*,#13692,.T.);
#19953=ORIENTED_EDGE('',*,*,#13688,.T.);
#19954=ORIENTED_EDGE('',*,*,#13687,.T.);
#19955=ORIENTED_EDGE('',*,*,#13683,.T.);
#19956=ORIENTED_EDGE('',*,*,#13682,.T.);
#19957=ORIENTED_EDGE('',*,*,#13678,.T.);
#19958=ORIENTED_EDGE('',*,*,#13677,.T.);
#19959=ORIENTED_EDGE('',*,*,#13673,.T.);
#19960=ORIENTED_EDGE('',*,*,#13672,.T.);
#19961=ORIENTED_EDGE('',*,*,#13668,.T.);
#19962=ORIENTED_EDGE('',*,*,#13667,.T.);
#19963=ORIENTED_EDGE('',*,*,#13663,.T.);
#19964=ORIENTED_EDGE('',*,*,#13662,.T.);
#19965=ORIENTED_EDGE('',*,*,#13658,.T.);
#19966=ORIENTED_EDGE('',*,*,#13657,.T.);
#19967=ORIENTED_EDGE('',*,*,#13653,.T.);
#19968=ORIENTED_EDGE('',*,*,#13652,.T.);
#19969=ORIENTED_EDGE('',*,*,#13648,.T.);
#19970=ORIENTED_EDGE('',*,*,#13647,.T.);
#19971=ORIENTED_EDGE('',*,*,#13643,.T.);
#19972=ORIENTED_EDGE('',*,*,#13642,.T.);
#19973=ORIENTED_EDGE('',*,*,#13638,.T.);
#19974=ORIENTED_EDGE('',*,*,#13637,.T.);
#19975=ORIENTED_EDGE('',*,*,#13633,.T.);
#19976=ORIENTED_EDGE('',*,*,#13632,.T.);
#19977=ORIENTED_EDGE('',*,*,#13628,.T.);
#19978=ORIENTED_EDGE('',*,*,#13627,.T.);
#19979=ORIENTED_EDGE('',*,*,#13623,.T.);
#19980=ORIENTED_EDGE('',*,*,#13622,.T.);
#19981=ORIENTED_EDGE('',*,*,#13618,.T.);
#19982=ORIENTED_EDGE('',*,*,#13617,.T.);
#19983=ORIENTED_EDGE('',*,*,#13613,.T.);
#19984=ORIENTED_EDGE('',*,*,#13612,.T.);
#19985=ORIENTED_EDGE('',*,*,#13608,.T.);
#19986=ORIENTED_EDGE('',*,*,#13607,.T.);
#19987=ORIENTED_EDGE('',*,*,#13603,.T.);
#19988=ORIENTED_EDGE('',*,*,#13602,.T.);
#19989=ORIENTED_EDGE('',*,*,#13598,.T.);
#19990=ORIENTED_EDGE('',*,*,#13597,.T.);
#19991=ORIENTED_EDGE('',*,*,#14481,.F.);
#19992=ORIENTED_EDGE('',*,*,#13732,.F.);
#19993=ORIENTED_EDGE('',*,*,#13731,.F.);
#19994=ORIENTED_EDGE('',*,*,#13738,.F.);
#19995=ORIENTED_EDGE('',*,*,#13737,.F.);
#19996=ORIENTED_EDGE('',*,*,#13743,.F.);
#19997=ORIENTED_EDGE('',*,*,#13742,.F.);
#19998=ORIENTED_EDGE('',*,*,#13748,.F.);
#19999=ORIENTED_EDGE('',*,*,#13747,.F.);
#20000=ORIENTED_EDGE('',*,*,#13753,.F.);
#20001=ORIENTED_EDGE('',*,*,#13752,.F.);
#20002=ORIENTED_EDGE('',*,*,#13758,.F.);
#20003=ORIENTED_EDGE('',*,*,#13757,.F.);
#20004=ORIENTED_EDGE('',*,*,#13763,.F.);
#20005=ORIENTED_EDGE('',*,*,#13762,.F.);
#20006=ORIENTED_EDGE('',*,*,#13768,.F.);
#20007=ORIENTED_EDGE('',*,*,#13767,.F.);
#20008=ORIENTED_EDGE('',*,*,#13773,.F.);
#20009=ORIENTED_EDGE('',*,*,#13772,.F.);
#20010=ORIENTED_EDGE('',*,*,#13778,.F.);
#20011=ORIENTED_EDGE('',*,*,#13777,.F.);
#20012=ORIENTED_EDGE('',*,*,#13783,.F.);
#20013=ORIENTED_EDGE('',*,*,#13782,.F.);
#20014=ORIENTED_EDGE('',*,*,#13788,.F.);
#20015=ORIENTED_EDGE('',*,*,#13787,.F.);
#20016=ORIENTED_EDGE('',*,*,#13793,.F.);
#20017=ORIENTED_EDGE('',*,*,#13792,.F.);
#20018=ORIENTED_EDGE('',*,*,#13798,.F.);
#20019=ORIENTED_EDGE('',*,*,#13797,.F.);
#20020=ORIENTED_EDGE('',*,*,#13803,.F.);
#20021=ORIENTED_EDGE('',*,*,#13802,.F.);
#20022=ORIENTED_EDGE('',*,*,#13808,.F.);
#20023=ORIENTED_EDGE('',*,*,#13807,.F.);
#20024=ORIENTED_EDGE('',*,*,#13813,.F.);
#20025=ORIENTED_EDGE('',*,*,#13812,.F.);
#20026=ORIENTED_EDGE('',*,*,#13818,.F.);
#20027=ORIENTED_EDGE('',*,*,#13817,.F.);
#20028=ORIENTED_EDGE('',*,*,#13823,.F.);
#20029=ORIENTED_EDGE('',*,*,#13822,.F.);
#20030=ORIENTED_EDGE('',*,*,#13828,.F.);
#20031=ORIENTED_EDGE('',*,*,#13827,.F.);
#20032=ORIENTED_EDGE('',*,*,#13833,.F.);
#20033=ORIENTED_EDGE('',*,*,#13832,.F.);
#20034=ORIENTED_EDGE('',*,*,#13838,.F.);
#20035=ORIENTED_EDGE('',*,*,#13837,.F.);
#20036=ORIENTED_EDGE('',*,*,#13843,.F.);
#20037=ORIENTED_EDGE('',*,*,#13842,.F.);
#20038=ORIENTED_EDGE('',*,*,#13848,.F.);
#20039=ORIENTED_EDGE('',*,*,#13847,.F.);
#20040=ORIENTED_EDGE('',*,*,#13853,.F.);
#20041=ORIENTED_EDGE('',*,*,#13852,.F.);
#20042=ORIENTED_EDGE('',*,*,#13858,.F.);
#20043=ORIENTED_EDGE('',*,*,#13857,.F.);
#20044=ORIENTED_EDGE('',*,*,#14386,.F.);
#20045=ORIENTED_EDGE('',*,*,#14385,.F.);
#20046=ORIENTED_EDGE('',*,*,#13866,.F.);
#20047=ORIENTED_EDGE('',*,*,#13865,.F.);
#20048=ORIENTED_EDGE('',*,*,#14496,.F.);
#20049=ORIENTED_EDGE('',*,*,#14014,.F.);
#20050=ORIENTED_EDGE('',*,*,#14377,.F.);
#20051=ORIENTED_EDGE('',*,*,#14376,.F.);
#20052=ORIENTED_EDGE('',*,*,#14012,.F.);
#20053=ORIENTED_EDGE('',*,*,#14009,.F.);
#20054=ORIENTED_EDGE('',*,*,#14008,.F.);
#20055=ORIENTED_EDGE('',*,*,#14004,.F.);
#20056=ORIENTED_EDGE('',*,*,#14003,.F.);
#20057=ORIENTED_EDGE('',*,*,#14000,.F.);
#20058=ORIENTED_EDGE('',*,*,#13999,.F.);
#20059=ORIENTED_EDGE('',*,*,#13995,.F.);
#20060=ORIENTED_EDGE('',*,*,#13992,.F.);
#20061=ORIENTED_EDGE('',*,*,#13991,.F.);
#20062=ORIENTED_EDGE('',*,*,#13987,.F.);
#20063=ORIENTED_EDGE('',*,*,#13984,.F.);
#20064=ORIENTED_EDGE('',*,*,#13983,.F.);
#20065=ORIENTED_EDGE('',*,*,#13979,.F.);
#20066=ORIENTED_EDGE('',*,*,#13978,.F.);
#20067=ORIENTED_EDGE('',*,*,#13975,.F.);
#20068=ORIENTED_EDGE('',*,*,#13974,.F.);
#20069=ORIENTED_EDGE('',*,*,#13970,.F.);
#20070=ORIENTED_EDGE('',*,*,#13966,.F.);
#20071=ORIENTED_EDGE('',*,*,#13965,.F.);
#20072=ORIENTED_EDGE('',*,*,#13961,.F.);
#20073=ORIENTED_EDGE('',*,*,#13958,.F.);
#20074=ORIENTED_EDGE('',*,*,#13957,.F.);
#20075=ORIENTED_EDGE('',*,*,#13953,.F.);
#20076=ORIENTED_EDGE('',*,*,#13952,.F.);
#20077=ORIENTED_EDGE('',*,*,#13949,.F.);
#20078=ORIENTED_EDGE('',*,*,#13948,.F.);
#20079=ORIENTED_EDGE('',*,*,#13944,.F.);
#20080=ORIENTED_EDGE('',*,*,#13940,.F.);
#20081=ORIENTED_EDGE('',*,*,#13939,.F.);
#20082=ORIENTED_EDGE('',*,*,#13935,.F.);
#20083=ORIENTED_EDGE('',*,*,#13932,.F.);
#20084=ORIENTED_EDGE('',*,*,#13931,.F.);
#20085=ORIENTED_EDGE('',*,*,#13927,.F.);
#20086=ORIENTED_EDGE('',*,*,#13924,.F.);
#20087=ORIENTED_EDGE('',*,*,#13923,.F.);
#20088=ORIENTED_EDGE('',*,*,#13919,.F.);
#20089=ORIENTED_EDGE('',*,*,#13915,.F.);
#20090=ORIENTED_EDGE('',*,*,#13914,.F.);
#20091=ORIENTED_EDGE('',*,*,#13910,.F.);
#20092=ORIENTED_EDGE('',*,*,#13907,.F.);
#20093=ORIENTED_EDGE('',*,*,#13906,.F.);
#20094=ORIENTED_EDGE('',*,*,#14480,.F.);
#20095=ORIENTED_EDGE('',*,*,#13904,.F.);
#20096=ORIENTED_EDGE('',*,*,#13903,.F.);
#20097=ORIENTED_EDGE('',*,*,#13909,.F.);
#20098=ORIENTED_EDGE('',*,*,#13913,.F.);
#20099=ORIENTED_EDGE('',*,*,#13912,.F.);
#20100=ORIENTED_EDGE('',*,*,#13918,.F.);
#20101=ORIENTED_EDGE('',*,*,#13917,.F.);
#20102=ORIENTED_EDGE('',*,*,#13922,.F.);
#20103=ORIENTED_EDGE('',*,*,#13921,.F.);
#20104=ORIENTED_EDGE('',*,*,#13926,.F.);
#20105=ORIENTED_EDGE('',*,*,#13930,.F.);
#20106=ORIENTED_EDGE('',*,*,#13929,.F.);
#20107=ORIENTED_EDGE('',*,*,#13934,.F.);
#20108=ORIENTED_EDGE('',*,*,#13938,.F.);
#20109=ORIENTED_EDGE('',*,*,#13937,.F.);
#20110=ORIENTED_EDGE('',*,*,#13943,.F.);
#20111=ORIENTED_EDGE('',*,*,#13942,.F.);
#20112=ORIENTED_EDGE('',*,*,#13947,.F.);
#20113=ORIENTED_EDGE('',*,*,#13946,.F.);
#20114=ORIENTED_EDGE('',*,*,#13951,.F.);
#20115=ORIENTED_EDGE('',*,*,#13956,.F.);
#20116=ORIENTED_EDGE('',*,*,#13955,.F.);
#20117=ORIENTED_EDGE('',*,*,#13960,.F.);
#20118=ORIENTED_EDGE('',*,*,#13964,.F.);
#20119=ORIENTED_EDGE('',*,*,#13963,.F.);
#20120=ORIENTED_EDGE('',*,*,#13969,.F.);
#20121=ORIENTED_EDGE('',*,*,#13968,.F.);
#20122=ORIENTED_EDGE('',*,*,#13973,.F.);
#20123=ORIENTED_EDGE('',*,*,#13972,.F.);
#20124=ORIENTED_EDGE('',*,*,#13977,.F.);
#20125=ORIENTED_EDGE('',*,*,#13982,.F.);
#20126=ORIENTED_EDGE('',*,*,#13981,.F.);
#20127=ORIENTED_EDGE('',*,*,#13986,.F.);
#20128=ORIENTED_EDGE('',*,*,#13990,.F.);
#20129=ORIENTED_EDGE('',*,*,#13989,.F.);
#20130=ORIENTED_EDGE('',*,*,#13994,.F.);
#20131=ORIENTED_EDGE('',*,*,#13998,.F.);
#20132=ORIENTED_EDGE('',*,*,#13997,.F.);
#20133=ORIENTED_EDGE('',*,*,#14002,.F.);
#20134=ORIENTED_EDGE('',*,*,#14007,.F.);
#20135=ORIENTED_EDGE('',*,*,#14006,.F.);
#20136=ORIENTED_EDGE('',*,*,#14011,.F.);
#20137=ORIENTED_EDGE('',*,*,#14375,.F.);
#20138=ORIENTED_EDGE('',*,*,#14374,.F.);
#20139=ORIENTED_EDGE('',*,*,#14016,.F.);
#20140=ORIENTED_EDGE('',*,*,#14497,.F.);
#20141=ORIENTED_EDGE('',*,*,#13863,.T.);
#20142=ORIENTED_EDGE('',*,*,#13862,.T.);
#20143=ORIENTED_EDGE('',*,*,#14388,.T.);
#20144=ORIENTED_EDGE('',*,*,#14387,.T.);
#20145=ORIENTED_EDGE('',*,*,#13860,.T.);
#20146=ORIENTED_EDGE('',*,*,#13859,.T.);
#20147=ORIENTED_EDGE('',*,*,#13855,.T.);
#20148=ORIENTED_EDGE('',*,*,#13854,.T.);
#20149=ORIENTED_EDGE('',*,*,#13850,.T.);
#20150=ORIENTED_EDGE('',*,*,#13849,.T.);
#20151=ORIENTED_EDGE('',*,*,#13845,.T.);
#20152=ORIENTED_EDGE('',*,*,#13844,.T.);
#20153=ORIENTED_EDGE('',*,*,#13840,.T.);
#20154=ORIENTED_EDGE('',*,*,#13839,.T.);
#20155=ORIENTED_EDGE('',*,*,#13835,.T.);
#20156=ORIENTED_EDGE('',*,*,#13834,.T.);
#20157=ORIENTED_EDGE('',*,*,#13830,.T.);
#20158=ORIENTED_EDGE('',*,*,#13829,.T.);
#20159=ORIENTED_EDGE('',*,*,#13825,.T.);
#20160=ORIENTED_EDGE('',*,*,#13824,.T.);
#20161=ORIENTED_EDGE('',*,*,#13820,.T.);
#20162=ORIENTED_EDGE('',*,*,#13819,.T.);
#20163=ORIENTED_EDGE('',*,*,#13815,.T.);
#20164=ORIENTED_EDGE('',*,*,#13814,.T.);
#20165=ORIENTED_EDGE('',*,*,#13810,.T.);
#20166=ORIENTED_EDGE('',*,*,#13809,.T.);
#20167=ORIENTED_EDGE('',*,*,#13805,.T.);
#20168=ORIENTED_EDGE('',*,*,#13804,.T.);
#20169=ORIENTED_EDGE('',*,*,#13800,.T.);
#20170=ORIENTED_EDGE('',*,*,#13799,.T.);
#20171=ORIENTED_EDGE('',*,*,#13795,.T.);
#20172=ORIENTED_EDGE('',*,*,#13794,.T.);
#20173=ORIENTED_EDGE('',*,*,#13790,.T.);
#20174=ORIENTED_EDGE('',*,*,#13789,.T.);
#20175=ORIENTED_EDGE('',*,*,#13785,.T.);
#20176=ORIENTED_EDGE('',*,*,#13784,.T.);
#20177=ORIENTED_EDGE('',*,*,#13780,.T.);
#20178=ORIENTED_EDGE('',*,*,#13779,.T.);
#20179=ORIENTED_EDGE('',*,*,#13775,.T.);
#20180=ORIENTED_EDGE('',*,*,#13774,.T.);
#20181=ORIENTED_EDGE('',*,*,#13770,.T.);
#20182=ORIENTED_EDGE('',*,*,#13769,.T.);
#20183=ORIENTED_EDGE('',*,*,#13765,.T.);
#20184=ORIENTED_EDGE('',*,*,#13764,.T.);
#20185=ORIENTED_EDGE('',*,*,#13760,.T.);
#20186=ORIENTED_EDGE('',*,*,#13759,.T.);
#20187=ORIENTED_EDGE('',*,*,#13755,.T.);
#20188=ORIENTED_EDGE('',*,*,#13754,.T.);
#20189=ORIENTED_EDGE('',*,*,#13750,.T.);
#20190=ORIENTED_EDGE('',*,*,#13749,.T.);
#20191=ORIENTED_EDGE('',*,*,#13745,.T.);
#20192=ORIENTED_EDGE('',*,*,#13744,.T.);
#20193=ORIENTED_EDGE('',*,*,#13740,.T.);
#20194=ORIENTED_EDGE('',*,*,#13739,.T.);
#20195=ORIENTED_EDGE('',*,*,#13735,.T.);
#20196=ORIENTED_EDGE('',*,*,#13734,.T.);
#20197=ORIENTED_EDGE('',*,*,#14498,.F.);
#20198=ORIENTED_EDGE('',*,*,#14499,.T.);
#20199=ORIENTED_EDGE('',*,*,#14500,.F.);
#20200=ORIENTED_EDGE('',*,*,#14501,.F.);
#20201=ORIENTED_EDGE('',*,*,#14502,.F.);
#20202=ORIENTED_EDGE('',*,*,#14501,.T.);
#20203=ORIENTED_EDGE('',*,*,#14503,.F.);
#20204=ORIENTED_EDGE('',*,*,#14504,.F.);
#20205=ORIENTED_EDGE('',*,*,#14505,.F.);
#20206=ORIENTED_EDGE('',*,*,#14504,.T.);
#20207=ORIENTED_EDGE('',*,*,#14506,.F.);
#20208=ORIENTED_EDGE('',*,*,#14507,.F.);
#20209=ORIENTED_EDGE('',*,*,#14508,.F.);
#20210=ORIENTED_EDGE('',*,*,#14507,.T.);
#20211=ORIENTED_EDGE('',*,*,#14509,.F.);
#20212=ORIENTED_EDGE('',*,*,#14510,.F.);
#20213=ORIENTED_EDGE('',*,*,#14511,.F.);
#20214=ORIENTED_EDGE('',*,*,#14510,.T.);
#20215=ORIENTED_EDGE('',*,*,#14512,.F.);
#20216=ORIENTED_EDGE('',*,*,#14513,.F.);
#20217=ORIENTED_EDGE('',*,*,#14514,.F.);
#20218=ORIENTED_EDGE('',*,*,#14513,.T.);
#20219=ORIENTED_EDGE('',*,*,#14515,.F.);
#20220=ORIENTED_EDGE('',*,*,#14516,.F.);
#20221=ORIENTED_EDGE('',*,*,#14517,.F.);
#20222=ORIENTED_EDGE('',*,*,#14516,.T.);
#20223=ORIENTED_EDGE('',*,*,#14518,.F.);
#20224=ORIENTED_EDGE('',*,*,#14499,.F.);
#20225=ORIENTED_EDGE('',*,*,#14519,.F.);
#20226=ORIENTED_EDGE('',*,*,#14520,.T.);
#20227=ORIENTED_EDGE('',*,*,#14521,.F.);
#20228=ORIENTED_EDGE('',*,*,#14520,.F.);
#20229=ORIENTED_EDGE('',*,*,#14519,.T.);
#20230=ORIENTED_EDGE('',*,*,#14518,.T.);
#20231=ORIENTED_EDGE('',*,*,#14515,.T.);
#20232=ORIENTED_EDGE('',*,*,#14512,.T.);
#20233=ORIENTED_EDGE('',*,*,#14509,.T.);
#20234=ORIENTED_EDGE('',*,*,#14506,.T.);
#20235=ORIENTED_EDGE('',*,*,#14503,.T.);
#20236=ORIENTED_EDGE('',*,*,#14500,.T.);
#20237=ORIENTED_EDGE('',*,*,#14522,.F.);
#20238=ORIENTED_EDGE('',*,*,#14523,.T.);
#20239=ORIENTED_EDGE('',*,*,#14524,.F.);
#20240=ORIENTED_EDGE('',*,*,#14525,.F.);
#20241=ORIENTED_EDGE('',*,*,#14526,.F.);
#20242=ORIENTED_EDGE('',*,*,#14525,.T.);
#20243=ORIENTED_EDGE('',*,*,#14527,.F.);
#20244=ORIENTED_EDGE('',*,*,#14528,.F.);
#20245=ORIENTED_EDGE('',*,*,#14529,.F.);
#20246=ORIENTED_EDGE('',*,*,#14528,.T.);
#20247=ORIENTED_EDGE('',*,*,#14530,.F.);
#20248=ORIENTED_EDGE('',*,*,#14531,.F.);
#20249=ORIENTED_EDGE('',*,*,#14532,.F.);
#20250=ORIENTED_EDGE('',*,*,#14531,.T.);
#20251=ORIENTED_EDGE('',*,*,#14533,.F.);
#20252=ORIENTED_EDGE('',*,*,#14453,.F.);
#20253=ORIENTED_EDGE('',*,*,#14534,.F.);
#20254=ORIENTED_EDGE('',*,*,#14455,.F.);
#20255=ORIENTED_EDGE('',*,*,#14535,.F.);
#20256=ORIENTED_EDGE('',*,*,#14523,.F.);
#20257=ORIENTED_EDGE('',*,*,#14535,.T.);
#20258=ORIENTED_EDGE('',*,*,#14454,.F.);
#20259=ORIENTED_EDGE('',*,*,#14533,.T.);
#20260=ORIENTED_EDGE('',*,*,#14530,.T.);
#20261=ORIENTED_EDGE('',*,*,#14527,.T.);
#20262=ORIENTED_EDGE('',*,*,#14524,.T.);
#20263=ORIENTED_EDGE('',*,*,#14489,.T.);
#20264=ORIENTED_EDGE('',*,*,#13869,.F.);
#20265=ORIENTED_EDGE('',*,*,#14487,.T.);
#20266=ORIENTED_EDGE('',*,*,#13316,.T.);
#20267=ORIENTED_EDGE('',*,*,#14536,.F.);
#20268=ORIENTED_EDGE('',*,*,#14537,.F.);
#20269=ORIENTED_EDGE('',*,*,#14538,.F.);
#20270=ORIENTED_EDGE('',*,*,#14539,.T.);
#20271=ORIENTED_EDGE('',*,*,#14540,.F.);
#20272=ORIENTED_EDGE('',*,*,#14541,.F.);
#20273=ORIENTED_EDGE('',*,*,#14542,.F.);
#20274=ORIENTED_EDGE('',*,*,#14541,.T.);
#20275=ORIENTED_EDGE('',*,*,#14543,.F.);
#20276=ORIENTED_EDGE('',*,*,#14544,.F.);
#20277=ORIENTED_EDGE('',*,*,#14545,.F.);
#20278=ORIENTED_EDGE('',*,*,#14544,.T.);
#20279=ORIENTED_EDGE('',*,*,#14546,.F.);
#20280=ORIENTED_EDGE('',*,*,#14547,.F.);
#20281=ORIENTED_EDGE('',*,*,#14548,.F.);
#20282=ORIENTED_EDGE('',*,*,#14547,.T.);
#20283=ORIENTED_EDGE('',*,*,#14549,.F.);
#20284=ORIENTED_EDGE('',*,*,#14550,.F.);
#20285=ORIENTED_EDGE('',*,*,#14551,.F.);
#20286=ORIENTED_EDGE('',*,*,#14550,.T.);
#20287=ORIENTED_EDGE('',*,*,#14552,.F.);
#20288=ORIENTED_EDGE('',*,*,#14553,.F.);
#20289=ORIENTED_EDGE('',*,*,#14554,.F.);
#20290=ORIENTED_EDGE('',*,*,#14553,.T.);
#20291=ORIENTED_EDGE('',*,*,#14555,.F.);
#20292=ORIENTED_EDGE('',*,*,#14556,.F.);
#20293=ORIENTED_EDGE('',*,*,#14557,.F.);
#20294=ORIENTED_EDGE('',*,*,#14556,.T.);
#20295=ORIENTED_EDGE('',*,*,#14558,.F.);
#20296=ORIENTED_EDGE('',*,*,#14539,.F.);
#20297=ORIENTED_EDGE('',*,*,#14559,.F.);
#20298=ORIENTED_EDGE('',*,*,#14560,.T.);
#20299=ORIENTED_EDGE('',*,*,#14561,.F.);
#20300=ORIENTED_EDGE('',*,*,#14560,.F.);
#20301=ORIENTED_EDGE('',*,*,#14559,.T.);
#20302=ORIENTED_EDGE('',*,*,#14558,.T.);
#20303=ORIENTED_EDGE('',*,*,#14555,.T.);
#20304=ORIENTED_EDGE('',*,*,#14552,.T.);
#20305=ORIENTED_EDGE('',*,*,#14549,.T.);
#20306=ORIENTED_EDGE('',*,*,#14546,.T.);
#20307=ORIENTED_EDGE('',*,*,#14543,.T.);
#20308=ORIENTED_EDGE('',*,*,#14540,.T.);
#20309=ORIENTED_EDGE('',*,*,#14538,.T.);
#20310=ORIENTED_EDGE('',*,*,#14542,.T.);
#20311=ORIENTED_EDGE('',*,*,#14545,.T.);
#20312=ORIENTED_EDGE('',*,*,#14548,.T.);
#20313=ORIENTED_EDGE('',*,*,#14551,.T.);
#20314=ORIENTED_EDGE('',*,*,#14554,.T.);
#20315=ORIENTED_EDGE('',*,*,#14557,.T.);
#20316=ORIENTED_EDGE('',*,*,#14498,.T.);
#20317=ORIENTED_EDGE('',*,*,#14502,.T.);
#20318=ORIENTED_EDGE('',*,*,#14505,.T.);
#20319=ORIENTED_EDGE('',*,*,#14508,.T.);
#20320=ORIENTED_EDGE('',*,*,#14511,.T.);
#20321=ORIENTED_EDGE('',*,*,#14514,.T.);
#20322=ORIENTED_EDGE('',*,*,#14517,.T.);
#20323=ORIENTED_EDGE('',*,*,#14562,.F.);
#20324=ORIENTED_EDGE('',*,*,#14563,.T.);
#20325=ORIENTED_EDGE('',*,*,#14536,.T.);
#20326=ORIENTED_EDGE('',*,*,#14563,.F.);
#20327=ORIENTED_EDGE('',*,*,#14562,.T.);
#20328=ORIENTED_EDGE('',*,*,#13883,.T.);
#20329=ORIENTED_EDGE('',*,*,#14384,.T.);
#20330=ORIENTED_EDGE('',*,*,#14488,.T.);
#20331=ORIENTED_EDGE('',*,*,#13301,.T.);
#20332=ORIENTED_EDGE('',*,*,#14486,.T.);
#20333=ORIENTED_EDGE('',*,*,#14564,.F.);
#20334=ORIENTED_EDGE('',*,*,#14565,.T.);
#20335=ORIENTED_EDGE('',*,*,#14537,.T.);
#20336=ORIENTED_EDGE('',*,*,#14565,.F.);
#20337=ORIENTED_EDGE('',*,*,#14564,.T.);
#20338=ORIENTED_EDGE('',*,*,#14566,.F.);
#20339=ORIENTED_EDGE('',*,*,#14567,.T.);
#20340=ORIENTED_EDGE('',*,*,#14568,.T.);
#20341=ORIENTED_EDGE('',*,*,#14569,.F.);
#20342=ORIENTED_EDGE('',*,*,#14570,.F.);
#20343=ORIENTED_EDGE('',*,*,#14571,.T.);
#20344=ORIENTED_EDGE('',*,*,#14572,.T.);
#20345=ORIENTED_EDGE('',*,*,#14567,.F.);
#20346=ORIENTED_EDGE('',*,*,#14573,.F.);
#20347=ORIENTED_EDGE('',*,*,#14574,.T.);
#20348=ORIENTED_EDGE('',*,*,#14575,.T.);
#20349=ORIENTED_EDGE('',*,*,#14571,.F.);
#20350=ORIENTED_EDGE('',*,*,#14576,.F.);
#20351=ORIENTED_EDGE('',*,*,#14463,.F.);
#20352=ORIENTED_EDGE('',*,*,#14577,.T.);
#20353=ORIENTED_EDGE('',*,*,#14574,.F.);
#20354=ORIENTED_EDGE('',*,*,#14578,.F.);
#20355=ORIENTED_EDGE('',*,*,#14569,.T.);
#20356=ORIENTED_EDGE('',*,*,#14579,.T.);
#20357=ORIENTED_EDGE('',*,*,#14461,.F.);
#20358=ORIENTED_EDGE('',*,*,#14579,.F.);
#20359=ORIENTED_EDGE('',*,*,#14568,.F.);
#20360=ORIENTED_EDGE('',*,*,#14572,.F.);
#20361=ORIENTED_EDGE('',*,*,#14575,.F.);
#20362=ORIENTED_EDGE('',*,*,#14577,.F.);
#20363=ORIENTED_EDGE('',*,*,#14462,.F.);
#20364=ORIENTED_EDGE('',*,*,#14485,.T.);
#20365=ORIENTED_EDGE('',*,*,#13899,.F.);
#20366=ORIENTED_EDGE('',*,*,#14483,.T.);
#20367=ORIENTED_EDGE('',*,*,#13296,.T.);
#20368=ORIENTED_EDGE('',*,*,#14580,.F.);
#20369=ORIENTED_EDGE('',*,*,#14581,.F.);
#20370=ORIENTED_EDGE('',*,*,#14582,.F.);
#20371=ORIENTED_EDGE('',*,*,#14583,.T.);
#20372=ORIENTED_EDGE('',*,*,#14584,.T.);
#20373=ORIENTED_EDGE('',*,*,#14585,.F.);
#20374=ORIENTED_EDGE('',*,*,#14586,.F.);
#20375=ORIENTED_EDGE('',*,*,#14587,.T.);
#20376=ORIENTED_EDGE('',*,*,#14588,.T.);
#20377=ORIENTED_EDGE('',*,*,#14583,.F.);
#20378=ORIENTED_EDGE('',*,*,#14589,.F.);
#20379=ORIENTED_EDGE('',*,*,#14590,.T.);
#20380=ORIENTED_EDGE('',*,*,#14591,.T.);
#20381=ORIENTED_EDGE('',*,*,#14587,.F.);
#20382=ORIENTED_EDGE('',*,*,#14592,.F.);
#20383=ORIENTED_EDGE('',*,*,#14593,.T.);
#20384=ORIENTED_EDGE('',*,*,#14594,.T.);
#20385=ORIENTED_EDGE('',*,*,#14590,.F.);
#20386=ORIENTED_EDGE('',*,*,#14595,.F.);
#20387=ORIENTED_EDGE('',*,*,#14596,.T.);
#20388=ORIENTED_EDGE('',*,*,#14597,.T.);
#20389=ORIENTED_EDGE('',*,*,#14593,.F.);
#20390=ORIENTED_EDGE('',*,*,#14598,.F.);
#20391=ORIENTED_EDGE('',*,*,#14599,.T.);
#20392=ORIENTED_EDGE('',*,*,#14600,.T.);
#20393=ORIENTED_EDGE('',*,*,#14596,.F.);
#20394=ORIENTED_EDGE('',*,*,#14601,.F.);
#20395=ORIENTED_EDGE('',*,*,#14585,.T.);
#20396=ORIENTED_EDGE('',*,*,#14602,.T.);
#20397=ORIENTED_EDGE('',*,*,#14599,.F.);
#20398=ORIENTED_EDGE('',*,*,#14603,.F.);
#20399=ORIENTED_EDGE('',*,*,#14604,.T.);
#20400=ORIENTED_EDGE('',*,*,#14605,.T.);
#20401=ORIENTED_EDGE('',*,*,#14604,.F.);
#20402=ORIENTED_EDGE('',*,*,#14605,.F.);
#20403=ORIENTED_EDGE('',*,*,#14602,.F.);
#20404=ORIENTED_EDGE('',*,*,#14584,.F.);
#20405=ORIENTED_EDGE('',*,*,#14588,.F.);
#20406=ORIENTED_EDGE('',*,*,#14591,.F.);
#20407=ORIENTED_EDGE('',*,*,#14594,.F.);
#20408=ORIENTED_EDGE('',*,*,#14597,.F.);
#20409=ORIENTED_EDGE('',*,*,#14600,.F.);
#20410=ORIENTED_EDGE('',*,*,#14606,.F.);
#20411=ORIENTED_EDGE('',*,*,#14607,.T.);
#20412=ORIENTED_EDGE('',*,*,#14608,.T.);
#20413=ORIENTED_EDGE('',*,*,#14609,.F.);
#20414=ORIENTED_EDGE('',*,*,#14610,.F.);
#20415=ORIENTED_EDGE('',*,*,#14611,.T.);
#20416=ORIENTED_EDGE('',*,*,#14612,.T.);
#20417=ORIENTED_EDGE('',*,*,#14607,.F.);
#20418=ORIENTED_EDGE('',*,*,#14613,.F.);
#20419=ORIENTED_EDGE('',*,*,#14614,.T.);
#20420=ORIENTED_EDGE('',*,*,#14615,.T.);
#20421=ORIENTED_EDGE('',*,*,#14611,.F.);
#20422=ORIENTED_EDGE('',*,*,#14616,.F.);
#20423=ORIENTED_EDGE('',*,*,#14617,.T.);
#20424=ORIENTED_EDGE('',*,*,#14618,.T.);
#20425=ORIENTED_EDGE('',*,*,#14614,.F.);
#20426=ORIENTED_EDGE('',*,*,#14619,.F.);
#20427=ORIENTED_EDGE('',*,*,#14620,.T.);
#20428=ORIENTED_EDGE('',*,*,#14621,.T.);
#20429=ORIENTED_EDGE('',*,*,#14617,.F.);
#20430=ORIENTED_EDGE('',*,*,#14622,.F.);
#20431=ORIENTED_EDGE('',*,*,#14623,.T.);
#20432=ORIENTED_EDGE('',*,*,#14624,.T.);
#20433=ORIENTED_EDGE('',*,*,#14620,.F.);
#20434=ORIENTED_EDGE('',*,*,#14625,.F.);
#20435=ORIENTED_EDGE('',*,*,#14609,.T.);
#20436=ORIENTED_EDGE('',*,*,#14626,.T.);
#20437=ORIENTED_EDGE('',*,*,#14623,.F.);
#20438=ORIENTED_EDGE('',*,*,#14627,.F.);
#20439=ORIENTED_EDGE('',*,*,#14628,.T.);
#20440=ORIENTED_EDGE('',*,*,#14629,.T.);
#20441=ORIENTED_EDGE('',*,*,#14628,.F.);
#20442=ORIENTED_EDGE('',*,*,#14629,.F.);
#20443=ORIENTED_EDGE('',*,*,#14626,.F.);
#20444=ORIENTED_EDGE('',*,*,#14608,.F.);
#20445=ORIENTED_EDGE('',*,*,#14612,.F.);
#20446=ORIENTED_EDGE('',*,*,#14615,.F.);
#20447=ORIENTED_EDGE('',*,*,#14618,.F.);
#20448=ORIENTED_EDGE('',*,*,#14621,.F.);
#20449=ORIENTED_EDGE('',*,*,#14624,.F.);
#20450=ORIENTED_EDGE('',*,*,#14606,.T.);
#20451=ORIENTED_EDGE('',*,*,#14625,.T.);
#20452=ORIENTED_EDGE('',*,*,#14622,.T.);
#20453=ORIENTED_EDGE('',*,*,#14619,.T.);
#20454=ORIENTED_EDGE('',*,*,#14616,.T.);
#20455=ORIENTED_EDGE('',*,*,#14613,.T.);
#20456=ORIENTED_EDGE('',*,*,#14610,.T.);
#20457=ORIENTED_EDGE('',*,*,#14582,.T.);
#20458=ORIENTED_EDGE('',*,*,#14601,.T.);
#20459=ORIENTED_EDGE('',*,*,#14598,.T.);
#20460=ORIENTED_EDGE('',*,*,#14595,.T.);
#20461=ORIENTED_EDGE('',*,*,#14592,.T.);
#20462=ORIENTED_EDGE('',*,*,#14589,.T.);
#20463=ORIENTED_EDGE('',*,*,#14586,.T.);
#20464=ORIENTED_EDGE('',*,*,#14576,.T.);
#20465=ORIENTED_EDGE('',*,*,#14573,.T.);
#20466=ORIENTED_EDGE('',*,*,#14570,.T.);
#20467=ORIENTED_EDGE('',*,*,#14566,.T.);
#20468=ORIENTED_EDGE('',*,*,#14578,.T.);
#20469=ORIENTED_EDGE('',*,*,#14460,.F.);
#20470=ORIENTED_EDGE('',*,*,#14630,.F.);
#20471=ORIENTED_EDGE('',*,*,#14631,.F.);
#20472=ORIENTED_EDGE('',*,*,#14632,.T.);
#20473=ORIENTED_EDGE('',*,*,#14464,.F.);
#20474=ORIENTED_EDGE('',*,*,#14627,.T.);
#20475=ORIENTED_EDGE('',*,*,#14603,.T.);
#20476=ORIENTED_EDGE('',*,*,#13890,.F.);
#20477=ORIENTED_EDGE('',*,*,#14484,.T.);
#20478=ORIENTED_EDGE('',*,*,#13281,.T.);
#20479=ORIENTED_EDGE('',*,*,#14482,.T.);
#20480=ORIENTED_EDGE('',*,*,#13886,.F.);
#20481=ORIENTED_EDGE('',*,*,#14581,.T.);
#20482=ORIENTED_EDGE('',*,*,#14633,.T.);
#20483=ORIENTED_EDGE('',*,*,#14634,.T.);
#20484=ORIENTED_EDGE('',*,*,#14633,.F.);
#20485=ORIENTED_EDGE('',*,*,#14634,.F.);
#20486=ORIENTED_EDGE('',*,*,#14580,.T.);
#20487=ORIENTED_EDGE('',*,*,#14635,.T.);
#20488=ORIENTED_EDGE('',*,*,#14636,.T.);
#20489=ORIENTED_EDGE('',*,*,#14635,.F.);
#20490=ORIENTED_EDGE('',*,*,#14636,.F.);
#20491=ORIENTED_EDGE('',*,*,#14472,.F.);
#20492=ORIENTED_EDGE('',*,*,#14637,.T.);
#20493=ORIENTED_EDGE('',*,*,#14638,.T.);
#20494=ORIENTED_EDGE('',*,*,#14637,.F.);
#20495=ORIENTED_EDGE('',*,*,#14638,.F.);
#20496=ORIENTED_EDGE('',*,*,#14473,.F.);
#20497=ORIENTED_EDGE('',*,*,#14639,.T.);
#20498=ORIENTED_EDGE('',*,*,#14640,.T.);
#20499=ORIENTED_EDGE('',*,*,#14639,.F.);
#20500=ORIENTED_EDGE('',*,*,#14640,.F.);
#20501=ORIENTED_EDGE('',*,*,#14427,.T.);
#20502=ORIENTED_EDGE('',*,*,#14641,.F.);
#20503=ORIENTED_EDGE('',*,*,#14642,.F.);
#20504=ORIENTED_EDGE('',*,*,#14442,.T.);
#20505=ORIENTED_EDGE('',*,*,#14430,.T.);
#20506=ORIENTED_EDGE('',*,*,#14440,.F.);
#20507=ORIENTED_EDGE('',*,*,#14643,.F.);
#20508=ORIENTED_EDGE('',*,*,#14641,.T.);
#20509=ORIENTED_EDGE('',*,*,#14644,.T.);
#20510=ORIENTED_EDGE('',*,*,#14438,.T.);
#20511=ORIENTED_EDGE('',*,*,#14471,.F.);
#20512=ORIENTED_EDGE('',*,*,#14645,.F.);
#20513=ORIENTED_EDGE('',*,*,#14646,.F.);
#20514=ORIENTED_EDGE('',*,*,#14645,.T.);
#20515=ORIENTED_EDGE('',*,*,#14470,.F.);
#20516=ORIENTED_EDGE('',*,*,#14647,.F.);
#20517=ORIENTED_EDGE('',*,*,#14648,.F.);
#20518=ORIENTED_EDGE('',*,*,#14647,.T.);
#20519=ORIENTED_EDGE('',*,*,#14469,.F.);
#20520=ORIENTED_EDGE('',*,*,#14649,.F.);
#20521=ORIENTED_EDGE('',*,*,#14650,.F.);
#20522=ORIENTED_EDGE('',*,*,#14649,.T.);
#20523=ORIENTED_EDGE('',*,*,#14468,.F.);
#20524=ORIENTED_EDGE('',*,*,#14651,.F.);
#20525=ORIENTED_EDGE('',*,*,#14652,.F.);
#20526=ORIENTED_EDGE('',*,*,#14651,.T.);
#20527=ORIENTED_EDGE('',*,*,#14467,.F.);
#20528=ORIENTED_EDGE('',*,*,#14653,.F.);
#20529=ORIENTED_EDGE('',*,*,#14654,.F.);
#20530=ORIENTED_EDGE('',*,*,#14653,.T.);
#20531=ORIENTED_EDGE('',*,*,#14466,.F.);
#20532=ORIENTED_EDGE('',*,*,#14655,.F.);
#20533=ORIENTED_EDGE('',*,*,#14656,.F.);
#20534=ORIENTED_EDGE('',*,*,#14655,.T.);
#20535=ORIENTED_EDGE('',*,*,#14465,.F.);
#20536=ORIENTED_EDGE('',*,*,#14632,.F.);
#20537=ORIENTED_EDGE('',*,*,#14657,.F.);
#20538=ORIENTED_EDGE('',*,*,#14630,.T.);
#20539=ORIENTED_EDGE('',*,*,#14459,.F.);
#20540=ORIENTED_EDGE('',*,*,#14658,.F.);
#20541=ORIENTED_EDGE('',*,*,#14659,.F.);
#20542=ORIENTED_EDGE('',*,*,#14658,.T.);
#20543=ORIENTED_EDGE('',*,*,#14458,.F.);
#20544=ORIENTED_EDGE('',*,*,#14660,.F.);
#20545=ORIENTED_EDGE('',*,*,#14661,.F.);
#20546=ORIENTED_EDGE('',*,*,#14660,.T.);
#20547=ORIENTED_EDGE('',*,*,#14457,.F.);
#20548=ORIENTED_EDGE('',*,*,#14662,.F.);
#20549=ORIENTED_EDGE('',*,*,#14532,.T.);
#20550=ORIENTED_EDGE('',*,*,#14452,.F.);
#20551=ORIENTED_EDGE('',*,*,#14663,.F.);
#20552=ORIENTED_EDGE('',*,*,#14664,.T.);
#20553=ORIENTED_EDGE('',*,*,#14662,.T.);
#20554=ORIENTED_EDGE('',*,*,#14456,.F.);
#20555=ORIENTED_EDGE('',*,*,#14534,.T.);
#20556=ORIENTED_EDGE('',*,*,#14522,.T.);
#20557=ORIENTED_EDGE('',*,*,#14526,.T.);
#20558=ORIENTED_EDGE('',*,*,#14529,.T.);
#20559=ORIENTED_EDGE('',*,*,#14561,.T.);
#20560=ORIENTED_EDGE('',*,*,#14521,.T.);
#20561=ORIENTED_EDGE('',*,*,#14665,.F.);
#20562=ORIENTED_EDGE('',*,*,#14663,.T.);
#20563=ORIENTED_EDGE('',*,*,#14451,.F.);
#20564=ORIENTED_EDGE('',*,*,#14666,.F.);
#20565=ORIENTED_EDGE('',*,*,#14667,.T.);
#20566=ORIENTED_EDGE('',*,*,#14666,.T.);
#20567=ORIENTED_EDGE('',*,*,#14450,.F.);
#20568=ORIENTED_EDGE('',*,*,#14668,.F.);
#20569=ORIENTED_EDGE('',*,*,#14669,.F.);
#20570=ORIENTED_EDGE('',*,*,#14668,.T.);
#20571=ORIENTED_EDGE('',*,*,#14449,.F.);
#20572=ORIENTED_EDGE('',*,*,#14670,.F.);
#20573=ORIENTED_EDGE('',*,*,#14671,.T.);
#20574=ORIENTED_EDGE('',*,*,#14670,.T.);
#20575=ORIENTED_EDGE('',*,*,#14448,.F.);
#20576=ORIENTED_EDGE('',*,*,#14672,.F.);
#20577=ORIENTED_EDGE('',*,*,#14673,.F.);
#20578=ORIENTED_EDGE('',*,*,#14672,.T.);
#20579=ORIENTED_EDGE('',*,*,#14447,.F.);
#20580=ORIENTED_EDGE('',*,*,#14674,.F.);
#20581=ORIENTED_EDGE('',*,*,#14675,.T.);
#20582=ORIENTED_EDGE('',*,*,#14674,.T.);
#20583=ORIENTED_EDGE('',*,*,#14446,.F.);
#20584=ORIENTED_EDGE('',*,*,#14676,.F.);
#20585=ORIENTED_EDGE('',*,*,#14677,.T.);
#20586=ORIENTED_EDGE('',*,*,#14676,.T.);
#20587=ORIENTED_EDGE('',*,*,#14445,.F.);
#20588=ORIENTED_EDGE('',*,*,#14678,.F.);
#20589=ORIENTED_EDGE('',*,*,#14416,.T.);
#20590=ORIENTED_EDGE('',*,*,#14679,.F.);
#20591=ORIENTED_EDGE('',*,*,#14680,.T.);
#20592=ORIENTED_EDGE('',*,*,#14678,.T.);
#20593=ORIENTED_EDGE('',*,*,#14444,.F.);
#20594=ORIENTED_EDGE('',*,*,#14415,.T.);
#20595=ORIENTED_EDGE('',*,*,#14419,.T.);
#20596=ORIENTED_EDGE('',*,*,#14436,.F.);
#20597=ORIENTED_EDGE('',*,*,#14681,.F.);
#20598=ORIENTED_EDGE('',*,*,#14679,.T.);
#20599=ORIENTED_EDGE('',*,*,#14681,.T.);
#20600=ORIENTED_EDGE('',*,*,#14435,.F.);
#20601=ORIENTED_EDGE('',*,*,#14443,.T.);
#20602=ORIENTED_EDGE('',*,*,#14642,.T.);
#20603=ORIENTED_EDGE('',*,*,#14643,.T.);
#20604=ORIENTED_EDGE('',*,*,#14439,.T.);
#20605=ORIENTED_EDGE('',*,*,#14644,.F.);
#20606=ORIENTED_EDGE('',*,*,#14646,.T.);
#20607=ORIENTED_EDGE('',*,*,#14648,.T.);
#20608=ORIENTED_EDGE('',*,*,#14650,.T.);
#20609=ORIENTED_EDGE('',*,*,#14652,.T.);
#20610=ORIENTED_EDGE('',*,*,#14654,.T.);
#20611=ORIENTED_EDGE('',*,*,#14656,.T.);
#20612=ORIENTED_EDGE('',*,*,#14631,.T.);
#20613=ORIENTED_EDGE('',*,*,#14657,.T.);
#20614=ORIENTED_EDGE('',*,*,#14659,.T.);
#20615=ORIENTED_EDGE('',*,*,#14661,.T.);
#20616=ORIENTED_EDGE('',*,*,#14664,.F.);
#20617=ORIENTED_EDGE('',*,*,#14665,.T.);
#20618=ORIENTED_EDGE('',*,*,#14667,.F.);
#20619=ORIENTED_EDGE('',*,*,#14669,.T.);
#20620=ORIENTED_EDGE('',*,*,#14671,.F.);
#20621=ORIENTED_EDGE('',*,*,#14673,.T.);
#20622=ORIENTED_EDGE('',*,*,#14675,.F.);
#20623=ORIENTED_EDGE('',*,*,#14677,.F.);
#20624=ORIENTED_EDGE('',*,*,#14680,.F.);
#20625=ORIENTED_EDGE('',*,*,#14491,.T.);
#20626=ORIENTED_EDGE('',*,*,#14360,.T.);
#20627=ORIENTED_EDGE('',*,*,#14490,.T.);
#20628=ORIENTED_EDGE('',*,*,#13453,.T.);
#20629=ORIENTED_EDGE('',*,*,#14493,.T.);
#20630=ORIENTED_EDGE('',*,*,#14245,.T.);
#20631=ORIENTED_EDGE('',*,*,#14492,.T.);
#20632=ORIENTED_EDGE('',*,*,#13590,.T.);
#20633=ORIENTED_EDGE('',*,*,#14495,.T.);
#20634=ORIENTED_EDGE('',*,*,#14130,.T.);
#20635=ORIENTED_EDGE('',*,*,#14494,.T.);
#20636=ORIENTED_EDGE('',*,*,#13727,.T.);
#20637=ORIENTED_EDGE('',*,*,#14497,.T.);
#20638=ORIENTED_EDGE('',*,*,#14015,.T.);
#20639=ORIENTED_EDGE('',*,*,#14496,.T.);
#20640=ORIENTED_EDGE('',*,*,#13864,.T.);
#26372=PLANE('',#28546);
#26373=PLANE('',#28550);
#26374=PLANE('',#28555);
#26375=PLANE('',#28559);
#26376=PLANE('',#28564);
#26377=PLANE('',#28565);
#26378=PLANE('',#28566);
#26379=PLANE('',#28567);
#26380=PLANE('',#28568);
#26381=PLANE('',#28581);
#26382=PLANE('',#28582);
#26383=PLANE('',#28583);
#26384=PLANE('',#28584);
#26385=PLANE('',#28585);
#26386=PLANE('',#28586);
#26387=PLANE('',#28587);
#26388=PLANE('',#28591);
#26389=PLANE('',#28595);
#26390=PLANE('',#28599);
#26391=PLANE('',#28600);
#26392=PLANE('',#28601);
#26393=PLANE('',#28604);
#26394=PLANE('',#28605);
#26395=PLANE('',#28606);
#26396=PLANE('',#28607);
#26397=PLANE('',#28608);
#26398=PLANE('',#28609);
#26399=PLANE('',#28610);
#26400=PLANE('',#28614);
#26401=PLANE('',#28615);
#26402=PLANE('',#28616);
#26403=PLANE('',#28619);
#26404=PLANE('',#28620);
#26405=PLANE('',#28623);
#26406=PLANE('',#28627);
#26407=PLANE('',#28631);
#26408=PLANE('',#28632);
#26409=PLANE('',#28633);
#26410=PLANE('',#28636);
#26411=PLANE('',#28637);
#26412=PLANE('',#28638);
#26413=PLANE('',#28639);
#26414=PLANE('',#28640);
#26415=PLANE('',#28641);
#26416=PLANE('',#28642);
#26417=PLANE('',#28646);
#26418=PLANE('',#28647);
#26419=PLANE('',#28648);
#26420=PLANE('',#28649);
#26421=PLANE('',#28650);
#26422=PLANE('',#28651);
#26423=PLANE('',#28652);
#26424=PLANE('',#28653);
#26425=PLANE('',#28657);
#26426=PLANE('',#28658);
#26427=PLANE('',#28659);
#26428=PLANE('',#28660);
#26429=PLANE('',#28661);
#26430=PLANE('',#28664);
#26431=PLANE('',#28667);
#26432=PLANE('',#28670);
#26433=PLANE('',#28673);
#26434=PLANE('',#28674);
#26435=PLANE('',#28679);
#26436=PLANE('',#28682);
#26437=PLANE('',#28685);
#26438=PLANE('',#28690);
#26439=PLANE('',#28693);
#26440=PLANE('',#28696);
#26441=PLANE('',#28699);
#26442=PLANE('',#28702);
#26443=PLANE('',#28705);
#26444=PLANE('',#28708);
#26822=ADVANCED_FACE('',(#3019),#2173,.F.);
#26823=ADVANCED_FACE('',(#3020),#2174,.F.);
#26824=ADVANCED_FACE('',(#3021),#2175,.F.);
#26825=ADVANCED_FACE('',(#3022),#2176,.F.);
#26826=ADVANCED_FACE('',(#3023),#2177,.F.);
#26827=ADVANCED_FACE('',(#3024),#2178,.F.);
#26828=ADVANCED_FACE('',(#3025),#2179,.F.);
#26829=ADVANCED_FACE('',(#3026),#2180,.F.);
#26830=ADVANCED_FACE('',(#3027),#2181,.F.);
#26831=ADVANCED_FACE('',(#3028),#2182,.F.);
#26832=ADVANCED_FACE('',(#3029),#2183,.F.);
#26833=ADVANCED_FACE('',(#3030),#2184,.F.);
#26834=ADVANCED_FACE('',(#3031),#2185,.F.);
#26835=ADVANCED_FACE('',(#3032),#2186,.F.);
#26836=ADVANCED_FACE('',(#3033),#2187,.F.);
#26837=ADVANCED_FACE('',(#3034),#2188,.F.);
#26838=ADVANCED_FACE('',(#3035),#2189,.F.);
#26839=ADVANCED_FACE('',(#3036),#2190,.F.);
#26840=ADVANCED_FACE('',(#3037),#2191,.F.);
#26841=ADVANCED_FACE('',(#3038),#2192,.F.);
#26842=ADVANCED_FACE('',(#3039),#2193,.F.);
#26843=ADVANCED_FACE('',(#3040),#2194,.F.);
#26844=ADVANCED_FACE('',(#3041),#2195,.F.);
#26845=ADVANCED_FACE('',(#3042),#2196,.F.);
#26846=ADVANCED_FACE('',(#3043),#2197,.F.);
#26847=ADVANCED_FACE('',(#3044),#2198,.F.);
#26848=ADVANCED_FACE('',(#3045),#2199,.F.);
#26849=ADVANCED_FACE('',(#3046),#2200,.F.);
#26850=ADVANCED_FACE('',(#3047),#2201,.F.);
#26851=ADVANCED_FACE('',(#3048),#2202,.F.);
#26852=ADVANCED_FACE('',(#3049),#2203,.F.);
#26853=ADVANCED_FACE('',(#3050),#2204,.F.);
#26854=ADVANCED_FACE('',(#3051),#2205,.F.);
#26855=ADVANCED_FACE('',(#3052),#2206,.F.);
#26856=ADVANCED_FACE('',(#3053),#2207,.F.);
#26857=ADVANCED_FACE('',(#3054),#2208,.F.);
#26858=ADVANCED_FACE('',(#3055),#2209,.F.);
#26859=ADVANCED_FACE('',(#3056),#2210,.F.);
#26860=ADVANCED_FACE('',(#3057),#2211,.F.);
#26861=ADVANCED_FACE('',(#3058),#2212,.F.);
#26862=ADVANCED_FACE('',(#3059),#2213,.F.);
#26863=ADVANCED_FACE('',(#3060),#2214,.F.);
#26864=ADVANCED_FACE('',(#3061),#2215,.F.);
#26865=ADVANCED_FACE('',(#3062),#2216,.F.);
#26866=ADVANCED_FACE('',(#3063),#2217,.F.);
#26867=ADVANCED_FACE('',(#3064),#2218,.F.);
#26868=ADVANCED_FACE('',(#3065),#2219,.F.);
#26869=ADVANCED_FACE('',(#3066),#2220,.F.);
#26870=ADVANCED_FACE('',(#3067),#2221,.F.);
#26871=ADVANCED_FACE('',(#3068),#2222,.F.);
#26872=ADVANCED_FACE('',(#3069),#2223,.F.);
#26873=ADVANCED_FACE('',(#3070),#2224,.F.);
#26874=ADVANCED_FACE('',(#3071),#2225,.F.);
#26875=ADVANCED_FACE('',(#3072),#2226,.F.);
#26876=ADVANCED_FACE('',(#3073),#2227,.F.);
#26877=ADVANCED_FACE('',(#3074),#2228,.F.);
#26878=ADVANCED_FACE('',(#3075),#2229,.F.);
#26879=ADVANCED_FACE('',(#3076),#2230,.F.);
#26880=ADVANCED_FACE('',(#3077),#2231,.F.);
#26881=ADVANCED_FACE('',(#3078),#2232,.F.);
#26882=ADVANCED_FACE('',(#3079),#2233,.F.);
#26883=ADVANCED_FACE('',(#3080),#2234,.F.);
#26884=ADVANCED_FACE('',(#3081),#2235,.F.);
#26885=ADVANCED_FACE('',(#3082),#2236,.F.);
#26886=ADVANCED_FACE('',(#3083),#2237,.F.);
#26887=ADVANCED_FACE('',(#3084),#2238,.F.);
#26888=ADVANCED_FACE('',(#3085),#2239,.F.);
#26889=ADVANCED_FACE('',(#3086),#2240,.F.);
#26890=ADVANCED_FACE('',(#3087),#2241,.F.);
#26891=ADVANCED_FACE('',(#3088),#2242,.F.);
#26892=ADVANCED_FACE('',(#3089),#2243,.F.);
#26893=ADVANCED_FACE('',(#3090),#2244,.F.);
#26894=ADVANCED_FACE('',(#3091),#2245,.F.);
#26895=ADVANCED_FACE('',(#3092),#2246,.F.);
#26896=ADVANCED_FACE('',(#3093),#2247,.F.);
#26897=ADVANCED_FACE('',(#3094),#2248,.F.);
#26898=ADVANCED_FACE('',(#3095),#2249,.F.);
#26899=ADVANCED_FACE('',(#3096),#2250,.F.);
#26900=ADVANCED_FACE('',(#3097),#2251,.F.);
#26901=ADVANCED_FACE('',(#3098),#2252,.F.);
#26902=ADVANCED_FACE('',(#3099),#2253,.F.);
#26903=ADVANCED_FACE('',(#3100),#2254,.F.);
#26904=ADVANCED_FACE('',(#3101),#2255,.F.);
#26905=ADVANCED_FACE('',(#3102),#2256,.F.);
#26906=ADVANCED_FACE('',(#3103),#2257,.F.);
#26907=ADVANCED_FACE('',(#3104),#2258,.F.);
#26908=ADVANCED_FACE('',(#3105),#2259,.F.);
#26909=ADVANCED_FACE('',(#3106),#2260,.F.);
#26910=ADVANCED_FACE('',(#3107),#2261,.F.);
#26911=ADVANCED_FACE('',(#3108),#2262,.F.);
#26912=ADVANCED_FACE('',(#3109),#2263,.F.);
#26913=ADVANCED_FACE('',(#3110),#2264,.F.);
#26914=ADVANCED_FACE('',(#3111),#2265,.F.);
#26915=ADVANCED_FACE('',(#3112),#2266,.F.);
#26916=ADVANCED_FACE('',(#3113),#2267,.F.);
#26917=ADVANCED_FACE('',(#3114),#2268,.F.);
#26918=ADVANCED_FACE('',(#3115),#2269,.F.);
#26919=ADVANCED_FACE('',(#3116),#2270,.F.);
#26920=ADVANCED_FACE('',(#3117),#2271,.F.);
#26921=ADVANCED_FACE('',(#3118),#2272,.F.);
#26922=ADVANCED_FACE('',(#3119),#2273,.F.);
#26923=ADVANCED_FACE('',(#3120),#2274,.F.);
#26924=ADVANCED_FACE('',(#3121),#2275,.F.);
#26925=ADVANCED_FACE('',(#3122),#2276,.F.);
#26926=ADVANCED_FACE('',(#3123),#2277,.F.);
#26927=ADVANCED_FACE('',(#3124),#2278,.F.);
#26928=ADVANCED_FACE('',(#3125),#2279,.F.);
#26929=ADVANCED_FACE('',(#3126),#2280,.F.);
#26930=ADVANCED_FACE('',(#3127),#2281,.F.);
#26931=ADVANCED_FACE('',(#3128),#2282,.F.);
#26932=ADVANCED_FACE('',(#3129),#2283,.F.);
#26933=ADVANCED_FACE('',(#3130),#2284,.F.);
#26934=ADVANCED_FACE('',(#3131),#2285,.F.);
#26935=ADVANCED_FACE('',(#3132),#2286,.F.);
#26936=ADVANCED_FACE('',(#3133),#2287,.F.);
#26937=ADVANCED_FACE('',(#3134),#2288,.F.);
#26938=ADVANCED_FACE('',(#3135),#2289,.F.);
#26939=ADVANCED_FACE('',(#3136),#2290,.F.);
#26940=ADVANCED_FACE('',(#3137),#2291,.F.);
#26941=ADVANCED_FACE('',(#3138),#2292,.F.);
#26942=ADVANCED_FACE('',(#3139),#2293,.F.);
#26943=ADVANCED_FACE('',(#3140),#2294,.F.);
#26944=ADVANCED_FACE('',(#3141),#2295,.F.);
#26945=ADVANCED_FACE('',(#3142),#2296,.F.);
#26946=ADVANCED_FACE('',(#3143),#2297,.F.);
#26947=ADVANCED_FACE('',(#3144),#2298,.F.);
#26948=ADVANCED_FACE('',(#3145),#2299,.F.);
#26949=ADVANCED_FACE('',(#3146),#2300,.F.);
#26950=ADVANCED_FACE('',(#3147),#2301,.F.);
#26951=ADVANCED_FACE('',(#3148),#2302,.F.);
#26952=ADVANCED_FACE('',(#3149),#2303,.F.);
#26953=ADVANCED_FACE('',(#3150),#2304,.F.);
#26954=ADVANCED_FACE('',(#3151),#2305,.F.);
#26955=ADVANCED_FACE('',(#3152),#2306,.F.);
#26956=ADVANCED_FACE('',(#3153),#2307,.F.);
#26957=ADVANCED_FACE('',(#3154),#2308,.F.);
#26958=ADVANCED_FACE('',(#3155),#2309,.F.);
#26959=ADVANCED_FACE('',(#3156),#2310,.F.);
#26960=ADVANCED_FACE('',(#3157),#2311,.F.);
#26961=ADVANCED_FACE('',(#3158),#2312,.F.);
#26962=ADVANCED_FACE('',(#3159),#2313,.F.);
#26963=ADVANCED_FACE('',(#3160),#2314,.F.);
#26964=ADVANCED_FACE('',(#3161),#2315,.F.);
#26965=ADVANCED_FACE('',(#3162),#2316,.F.);
#26966=ADVANCED_FACE('',(#3163),#2317,.F.);
#26967=ADVANCED_FACE('',(#3164),#2318,.F.);
#26968=ADVANCED_FACE('',(#3165),#2319,.F.);
#26969=ADVANCED_FACE('',(#3166),#2320,.F.);
#26970=ADVANCED_FACE('',(#3167),#2321,.F.);
#26971=ADVANCED_FACE('',(#3168),#2322,.F.);
#26972=ADVANCED_FACE('',(#3169),#2323,.F.);
#26973=ADVANCED_FACE('',(#3170),#2324,.F.);
#26974=ADVANCED_FACE('',(#3171),#2325,.F.);
#26975=ADVANCED_FACE('',(#3172),#2326,.F.);
#26976=ADVANCED_FACE('',(#3173),#2327,.F.);
#26977=ADVANCED_FACE('',(#3174),#2328,.F.);
#26978=ADVANCED_FACE('',(#3175),#2329,.F.);
#26979=ADVANCED_FACE('',(#3176),#2330,.F.);
#26980=ADVANCED_FACE('',(#3177),#2331,.F.);
#26981=ADVANCED_FACE('',(#3178),#2332,.F.);
#26982=ADVANCED_FACE('',(#3179),#2333,.F.);
#26983=ADVANCED_FACE('',(#3180),#2334,.F.);
#26984=ADVANCED_FACE('',(#3181),#2335,.F.);
#26985=ADVANCED_FACE('',(#3182),#2336,.F.);
#26986=ADVANCED_FACE('',(#3183),#2337,.F.);
#26987=ADVANCED_FACE('',(#3184),#2338,.F.);
#26988=ADVANCED_FACE('',(#3185),#2339,.F.);
#26989=ADVANCED_FACE('',(#3186),#2340,.F.);
#26990=ADVANCED_FACE('',(#3187),#2341,.F.);
#26991=ADVANCED_FACE('',(#3188),#2342,.F.);
#26992=ADVANCED_FACE('',(#3189),#2343,.F.);
#26993=ADVANCED_FACE('',(#3190),#2344,.F.);
#26994=ADVANCED_FACE('',(#3191),#2345,.F.);
#26995=ADVANCED_FACE('',(#3192),#2346,.F.);
#26996=ADVANCED_FACE('',(#3193),#2347,.F.);
#26997=ADVANCED_FACE('',(#3194),#2348,.F.);
#26998=ADVANCED_FACE('',(#3195),#2349,.F.);
#26999=ADVANCED_FACE('',(#3196),#2350,.F.);
#27000=ADVANCED_FACE('',(#3197),#2351,.F.);
#27001=ADVANCED_FACE('',(#3198),#2352,.F.);
#27002=ADVANCED_FACE('',(#3199),#2353,.F.);
#27003=ADVANCED_FACE('',(#3200),#2354,.F.);
#27004=ADVANCED_FACE('',(#3201),#2355,.F.);
#27005=ADVANCED_FACE('',(#3202),#2356,.F.);
#27006=ADVANCED_FACE('',(#3203),#2357,.F.);
#27007=ADVANCED_FACE('',(#3204),#2358,.F.);
#27008=ADVANCED_FACE('',(#3205),#2359,.F.);
#27009=ADVANCED_FACE('',(#3206),#2360,.F.);
#27010=ADVANCED_FACE('',(#3207),#2361,.F.);
#27011=ADVANCED_FACE('',(#3208),#2362,.F.);
#27012=ADVANCED_FACE('',(#3209),#2363,.F.);
#27013=ADVANCED_FACE('',(#3210),#2364,.F.);
#27014=ADVANCED_FACE('',(#3211),#2365,.F.);
#27015=ADVANCED_FACE('',(#3212),#2366,.F.);
#27016=ADVANCED_FACE('',(#3213),#2367,.F.);
#27017=ADVANCED_FACE('',(#3214),#2368,.F.);
#27018=ADVANCED_FACE('',(#3215),#2369,.F.);
#27019=ADVANCED_FACE('',(#3216),#2370,.F.);
#27020=ADVANCED_FACE('',(#3217),#2371,.F.);
#27021=ADVANCED_FACE('',(#3218),#2372,.F.);
#27022=ADVANCED_FACE('',(#3219),#2373,.F.);
#27023=ADVANCED_FACE('',(#3220),#2374,.F.);
#27024=ADVANCED_FACE('',(#3221),#2375,.F.);
#27025=ADVANCED_FACE('',(#3222),#2376,.F.);
#27026=ADVANCED_FACE('',(#3223),#2377,.F.);
#27027=ADVANCED_FACE('',(#3224),#2378,.F.);
#27028=ADVANCED_FACE('',(#3225),#2379,.F.);
#27029=ADVANCED_FACE('',(#3226),#2380,.F.);
#27030=ADVANCED_FACE('',(#3227),#2381,.F.);
#27031=ADVANCED_FACE('',(#3228),#2382,.F.);
#27032=ADVANCED_FACE('',(#3229),#2383,.F.);
#27033=ADVANCED_FACE('',(#3230),#2384,.F.);
#27034=ADVANCED_FACE('',(#3231),#2385,.F.);
#27035=ADVANCED_FACE('',(#3232),#2386,.F.);
#27036=ADVANCED_FACE('',(#3233),#2387,.F.);
#27037=ADVANCED_FACE('',(#3234),#2388,.F.);
#27038=ADVANCED_FACE('',(#3235),#2389,.F.);
#27039=ADVANCED_FACE('',(#3236),#2390,.F.);
#27040=ADVANCED_FACE('',(#3237),#2391,.F.);
#27041=ADVANCED_FACE('',(#3238),#2392,.F.);
#27042=ADVANCED_FACE('',(#3239),#2393,.F.);
#27043=ADVANCED_FACE('',(#3240),#2394,.F.);
#27044=ADVANCED_FACE('',(#3241),#2395,.F.);
#27045=ADVANCED_FACE('',(#3242),#2396,.F.);
#27046=ADVANCED_FACE('',(#3243),#2397,.F.);
#27047=ADVANCED_FACE('',(#3244),#2398,.F.);
#27048=ADVANCED_FACE('',(#3245),#2399,.F.);
#27049=ADVANCED_FACE('',(#3246),#2400,.F.);
#27050=ADVANCED_FACE('',(#3247),#2401,.F.);
#27051=ADVANCED_FACE('',(#3248),#2402,.F.);
#27052=ADVANCED_FACE('',(#3249),#2403,.F.);
#27053=ADVANCED_FACE('',(#3250),#2404,.F.);
#27054=ADVANCED_FACE('',(#3251),#2405,.F.);
#27055=ADVANCED_FACE('',(#3252),#2406,.F.);
#27056=ADVANCED_FACE('',(#3253),#2407,.F.);
#27057=ADVANCED_FACE('',(#3254),#2408,.F.);
#27058=ADVANCED_FACE('',(#3255),#2409,.F.);
#27059=ADVANCED_FACE('',(#3256),#2410,.F.);
#27060=ADVANCED_FACE('',(#3257),#2411,.F.);
#27061=ADVANCED_FACE('',(#3258),#2412,.F.);
#27062=ADVANCED_FACE('',(#3259),#2413,.F.);
#27063=ADVANCED_FACE('',(#3260),#2414,.F.);
#27064=ADVANCED_FACE('',(#3261),#2415,.F.);
#27065=ADVANCED_FACE('',(#3262),#2416,.F.);
#27066=ADVANCED_FACE('',(#3263),#2417,.F.);
#27067=ADVANCED_FACE('',(#3264),#26372,.T.);
#27068=ADVANCED_FACE('',(#3265),#2418,.F.);
#27069=ADVANCED_FACE('',(#3266),#26373,.T.);
#27070=ADVANCED_FACE('',(#3267),#2419,.F.);
#27071=ADVANCED_FACE('',(#3268),#26374,.T.);
#27072=ADVANCED_FACE('',(#3269),#2420,.F.);
#27073=ADVANCED_FACE('',(#3270),#26375,.T.);
#27074=ADVANCED_FACE('',(#3271),#2421,.F.);
#27075=ADVANCED_FACE('',(#3272),#26376,.T.);
#27076=ADVANCED_FACE('',(#3273),#26377,.T.);
#27077=ADVANCED_FACE('',(#3274),#26378,.T.);
#27078=ADVANCED_FACE('',(#3275),#26379,.T.);
#27079=ADVANCED_FACE('',(#3276,#173,#174,#175,#176,#177,#178,#179,#180,
#181),#26380,.F.);
#27080=ADVANCED_FACE('',(#3277),#149,.F.);
#27081=ADVANCED_FACE('',(#3278),#150,.F.);
#27082=ADVANCED_FACE('',(#3279),#151,.F.);
#27083=ADVANCED_FACE('',(#3280),#152,.F.);
#27084=ADVANCED_FACE('',(#3281),#153,.F.);
#27085=ADVANCED_FACE('',(#3282),#154,.F.);
#27086=ADVANCED_FACE('',(#3283),#155,.F.);
#27087=ADVANCED_FACE('',(#3284),#156,.F.);
#27088=ADVANCED_FACE('',(#3285),#157,.F.);
#27089=ADVANCED_FACE('',(#3286),#158,.F.);
#27090=ADVANCED_FACE('',(#3287),#159,.F.);
#27091=ADVANCED_FACE('',(#3288),#160,.F.);
#27092=ADVANCED_FACE('',(#3289),#26381,.T.);
#27093=ADVANCED_FACE('',(#3290),#26382,.T.);
#27094=ADVANCED_FACE('',(#3291),#26383,.T.);
#27095=ADVANCED_FACE('',(#3292),#26384,.T.);
#27096=ADVANCED_FACE('',(#3293),#26385,.T.);
#27097=ADVANCED_FACE('',(#3294),#26386,.T.);
#27098=ADVANCED_FACE('',(#3295),#26387,.T.);
#27099=ADVANCED_FACE('',(#3296),#2422,.F.);
#27100=ADVANCED_FACE('',(#3297,#182),#26388,.F.);
#27101=ADVANCED_FACE('',(#3298),#2423,.F.);
#27102=ADVANCED_FACE('',(#3299),#26389,.T.);
#27103=ADVANCED_FACE('',(#3300),#2424,.F.);
#27104=ADVANCED_FACE('',(#3301),#26390,.T.);
#27105=ADVANCED_FACE('',(#3302),#26391,.T.);
#27106=ADVANCED_FACE('',(#3303,#183,#184,#185),#26392,.F.);
#27107=ADVANCED_FACE('',(#3304),#26393,.T.);
#27108=ADVANCED_FACE('',(#3305),#26394,.T.);
#27109=ADVANCED_FACE('',(#3306),#26395,.T.);
#27110=ADVANCED_FACE('',(#3307),#26396,.T.);
#27111=ADVANCED_FACE('',(#3308),#26397,.T.);
#27112=ADVANCED_FACE('',(#3309),#26398,.T.);
#27113=ADVANCED_FACE('',(#3310),#26399,.T.);
#27114=ADVANCED_FACE('',(#3311),#2425,.F.);
#27115=ADVANCED_FACE('',(#3312,#186),#26400,.F.);
#27116=ADVANCED_FACE('',(#3313),#26401,.T.);
#27117=ADVANCED_FACE('',(#3314),#26402,.T.);
#27118=ADVANCED_FACE('',(#3315),#2426,.F.);
#27119=ADVANCED_FACE('',(#3316),#26403,.F.);
#27120=ADVANCED_FACE('',(#3317),#26404,.F.);
#27121=ADVANCED_FACE('',(#3318),#2427,.F.);
#27122=ADVANCED_FACE('',(#3319),#26405,.F.);
#27123=ADVANCED_FACE('',(#3320),#2428,.F.);
#27124=ADVANCED_FACE('',(#3321),#26406,.F.);
#27125=ADVANCED_FACE('',(#3322),#2429,.F.);
#27126=ADVANCED_FACE('',(#3323),#26407,.F.);
#27127=ADVANCED_FACE('',(#3324),#26408,.F.);
#27128=ADVANCED_FACE('',(#3325,#187,#188,#189),#26409,.T.);
#27129=ADVANCED_FACE('',(#3326),#26410,.F.);
#27130=ADVANCED_FACE('',(#3327),#26411,.F.);
#27131=ADVANCED_FACE('',(#3328),#26412,.F.);
#27132=ADVANCED_FACE('',(#3329),#26413,.F.);
#27133=ADVANCED_FACE('',(#3330),#26414,.F.);
#27134=ADVANCED_FACE('',(#3331),#26415,.F.);
#27135=ADVANCED_FACE('',(#3332),#26416,.F.);
#27136=ADVANCED_FACE('',(#3333),#2430,.F.);
#27137=ADVANCED_FACE('',(#3334,#190),#26417,.T.);
#27138=ADVANCED_FACE('',(#3335),#26418,.F.);
#27139=ADVANCED_FACE('',(#3336),#26419,.F.);
#27140=ADVANCED_FACE('',(#3337),#26420,.F.);
#27141=ADVANCED_FACE('',(#3338),#26421,.F.);
#27142=ADVANCED_FACE('',(#3339),#26422,.F.);
#27143=ADVANCED_FACE('',(#3340),#26423,.F.);
#27144=ADVANCED_FACE('',(#3341),#26424,.F.);
#27145=ADVANCED_FACE('',(#3342),#2431,.F.);
#27146=ADVANCED_FACE('',(#3343,#191),#26425,.T.);
#27147=ADVANCED_FACE('',(#3344),#26426,.T.);
#27148=ADVANCED_FACE('',(#3345),#26427,.T.);
#27149=ADVANCED_FACE('',(#3346,#192,#193),#26428,.T.);
#27150=ADVANCED_FACE('',(#3347),#26429,.T.);
#27151=ADVANCED_FACE('',(#3348),#2432,.F.);
#27152=ADVANCED_FACE('',(#3349),#26430,.T.);
#27153=ADVANCED_FACE('',(#3350),#2433,.F.);
#27154=ADVANCED_FACE('',(#3351),#26431,.T.);
#27155=ADVANCED_FACE('',(#3352),#2434,.F.);
#27156=ADVANCED_FACE('',(#3353),#26432,.T.);
#27157=ADVANCED_FACE('',(#3354),#2435,.F.);
#27158=ADVANCED_FACE('',(#3355),#26433,.T.);
#27159=ADVANCED_FACE('',(#3356),#26434,.T.);
#27160=ADVANCED_FACE('',(#3357),#2436,.T.);
#27161=ADVANCED_FACE('',(#3358),#2437,.F.);
#27162=ADVANCED_FACE('',(#3359),#26435,.T.);
#27163=ADVANCED_FACE('',(#3360),#2438,.T.);
#27164=ADVANCED_FACE('',(#3361),#26436,.T.);
#27165=ADVANCED_FACE('',(#3362),#2439,.T.);
#27166=ADVANCED_FACE('',(#3363),#26437,.T.);
#27167=ADVANCED_FACE('',(#3364),#2440,.T.);
#27168=ADVANCED_FACE('',(#3365),#2441,.T.);
#27169=ADVANCED_FACE('',(#3366),#26438,.T.);
#27170=ADVANCED_FACE('',(#3367),#2442,.T.);
#27171=ADVANCED_FACE('',(#3368,#194,#195),#26439,.T.);
#27172=ADVANCED_FACE('',(#3369),#2443,.T.);
#27173=ADVANCED_FACE('',(#3370),#26440,.T.);
#27174=ADVANCED_FACE('',(#3371),#2444,.T.);
#27175=ADVANCED_FACE('',(#3372),#26441,.T.);
#27176=ADVANCED_FACE('',(#3373),#2445,.T.);
#27177=ADVANCED_FACE('',(#3374),#26442,.T.);
#27178=ADVANCED_FACE('',(#3375),#2446,.F.);
#27179=ADVANCED_FACE('',(#3376),#26443,.T.);
#27180=ADVANCED_FACE('',(#3377),#2447,.T.);
#27181=ADVANCED_FACE('',(#3378,#196,#197,#198,#199),#26444,.T.);
#28082=CLOSED_SHELL('',(#26822,#26823,#26824,#26825,#26826,#26827,#26828,
#26829,#26830,#26831,#26832,#26833,#26834,#26835,#26836,#26837,#26838,#26839,
#26840,#26841,#26842,#26843,#26844,#26845,#26846,#26847,#26848,#26849,#26850,
#26851,#26852,#26853,#26854,#26855,#26856,#26857,#26858,#26859,#26860,#26861,
#26862,#26863,#26864,#26865,#26866,#26867,#26868,#26869,#26870,#26871,#26872,
#26873,#26874,#26875,#26876,#26877,#26878,#26879,#26880,#26881,#26882,#26883,
#26884,#26885,#26886,#26887,#26888,#26889,#26890,#26891,#26892,#26893,#26894,
#26895,#26896,#26897,#26898,#26899,#26900,#26901,#26902,#26903,#26904,#26905,
#26906,#26907,#26908,#26909,#26910,#26911,#26912,#26913,#26914,#26915,#26916,
#26917,#26918,#26919,#26920,#26921,#26922,#26923,#26924,#26925,#26926,#26927,
#26928,#26929,#26930,#26931,#26932,#26933,#26934,#26935,#26936,#26937,#26938,
#26939,#26940,#26941,#26942,#26943,#26944,#26945,#26946,#26947,#26948,#26949,
#26950,#26951,#26952,#26953,#26954,#26955,#26956,#26957,#26958,#26959,#26960,
#26961,#26962,#26963,#26964,#26965,#26966,#26967,#26968,#26969,#26970,#26971,
#26972,#26973,#26974,#26975,#26976,#26977,#26978,#26979,#26980,#26981,#26982,
#26983,#26984,#26985,#26986,#26987,#26988,#26989,#26990,#26991,#26992,#26993,
#26994,#26995,#26996,#26997,#26998,#26999,#27000,#27001,#27002,#27003,#27004,
#27005,#27006,#27007,#27008,#27009,#27010,#27011,#27012,#27013,#27014,#27015,
#27016,#27017,#27018,#27019,#27020,#27021,#27022,#27023,#27024,#27025,#27026,
#27027,#27028,#27029,#27030,#27031,#27032,#27033,#27034,#27035,#27036,#27037,
#27038,#27039,#27040,#27041,#27042,#27043,#27044,#27045,#27046,#27047,#27048,
#27049,#27050,#27051,#27052,#27053,#27054,#27055,#27056,#27057,#27058,#27059,
#27060,#27061,#27062,#27063,#27064,#27065,#27066,#27067,#27068,#27069,#27070,
#27071,#27072,#27073,#27074,#27075,#27076,#27077,#27078,#27079,#27080,#27081,
#27082,#27083,#27084,#27085,#27086,#27087,#27088,#27089,#27090,#27091,#27092,
#27093,#27094,#27095,#27096,#27097,#27098,#27099,#27100,#27101,#27102,#27103,
#27104,#27105,#27106,#27107,#27108,#27109,#27110,#27111,#27112,#27113,#27114,
#27115,#27116,#27117,#27118,#27119,#27120,#27121,#27122,#27123,#27124,#27125,
#27126,#27127,#27128,#27129,#27130,#27131,#27132,#27133,#27134,#27135,#27136,
#27137,#27138,#27139,#27140,#27141,#27142,#27143,#27144,#27145,#27146,#27147,
#27148,#27149,#27150,#27151,#27152,#27153,#27154,#27155,#27156,#27157,#27158,
#27159,#27160,#27161,#27162,#27163,#27164,#27165,#27166,#27167,#27168,#27169,
#27170,#27171,#27172,#27173,#27174,#27175,#27176,#27177,#27178,#27179,#27180,
#27181));
#28272=AXIS2_PLACEMENT_3D('',#36294,#30469,#30470);
#28273=AXIS2_PLACEMENT_3D('',#36295,#30471,#30472);
#28274=AXIS2_PLACEMENT_3D('',#36307,#30474,#30475);
#28275=AXIS2_PLACEMENT_3D('',#36381,#30476,#30477);
#28276=AXIS2_PLACEMENT_3D('',#36644,#30479,#30480);
#28277=AXIS2_PLACEMENT_3D('',#37042,#30482,#30483);
#28278=AXIS2_PLACEMENT_3D('',#37140,#30485,#30486);
#28279=AXIS2_PLACEMENT_3D('',#37218,#30487,#30488);
#28280=AXIS2_PLACEMENT_3D('',#37230,#30490,#30491);
#28281=AXIS2_PLACEMENT_3D('',#37304,#30492,#30493);
#28282=AXIS2_PLACEMENT_3D('',#37567,#30495,#30496);
#28283=AXIS2_PLACEMENT_3D('',#37965,#30498,#30499);
#28284=AXIS2_PLACEMENT_3D('',#38063,#30501,#30502);
#28285=AXIS2_PLACEMENT_3D('',#38141,#30503,#30504);
#28286=AXIS2_PLACEMENT_3D('',#38161,#30506,#30507);
#28287=AXIS2_PLACEMENT_3D('',#38229,#30508,#30509);
#28288=AXIS2_PLACEMENT_3D('',#38380,#30511,#30512);
#28289=AXIS2_PLACEMENT_3D('',#38713,#30514,#30515);
#28290=AXIS2_PLACEMENT_3D('',#38994,#30517,#30518);
#28291=AXIS2_PLACEMENT_3D('',#39330,#30520,#30521);
#28292=AXIS2_PLACEMENT_3D('',#39492,#30523,#30524);
#28293=AXIS2_PLACEMENT_3D('',#39762,#30526,#30527);
#28294=AXIS2_PLACEMENT_3D('',#40037,#30529,#30530);
#28295=AXIS2_PLACEMENT_3D('',#40371,#30532,#30533);
#28296=AXIS2_PLACEMENT_3D('',#40533,#30535,#30536);
#28297=AXIS2_PLACEMENT_3D('',#40800,#30538,#30539);
#28298=AXIS2_PLACEMENT_3D('',#41078,#30541,#30542);
#28299=AXIS2_PLACEMENT_3D('',#41411,#30544,#30545);
#28300=AXIS2_PLACEMENT_3D('',#41576,#30547,#30548);
#28301=AXIS2_PLACEMENT_3D('',#41845,#30550,#30551);
#28302=AXIS2_PLACEMENT_3D('',#42126,#30553,#30554);
#28303=AXIS2_PLACEMENT_3D('',#42459,#30556,#30557);
#28304=AXIS2_PLACEMENT_3D('',#42618,#30559,#30560);
#28305=AXIS2_PLACEMENT_3D('',#42888,#30562,#30563);
#28306=AXIS2_PLACEMENT_3D('',#43169,#30565,#30566);
#28307=AXIS2_PLACEMENT_3D('',#43500,#30568,#30569);
#28308=AXIS2_PLACEMENT_3D('',#43663,#30571,#30572);
#28309=AXIS2_PLACEMENT_3D('',#43929,#30574,#30575);
#28310=AXIS2_PLACEMENT_3D('',#44210,#30577,#30578);
#28311=AXIS2_PLACEMENT_3D('',#44543,#30580,#30581);
#28312=AXIS2_PLACEMENT_3D('',#44824,#30583,#30584);
#28313=AXIS2_PLACEMENT_3D('',#44842,#30586,#30587);
#28314=AXIS2_PLACEMENT_3D('',#44909,#30588,#30589);
#28315=AXIS2_PLACEMENT_3D('',#44929,#30591,#30592);
#28316=AXIS2_PLACEMENT_3D('',#44997,#30593,#30594);
#28317=AXIS2_PLACEMENT_3D('',#45148,#30596,#30597);
#28318=AXIS2_PLACEMENT_3D('',#45481,#30599,#30600);
#28319=AXIS2_PLACEMENT_3D('',#45762,#30602,#30603);
#28320=AXIS2_PLACEMENT_3D('',#46098,#30605,#30606);
#28321=AXIS2_PLACEMENT_3D('',#46260,#30608,#30609);
#28322=AXIS2_PLACEMENT_3D('',#46530,#30611,#30612);
#28323=AXIS2_PLACEMENT_3D('',#46805,#30614,#30615);
#28324=AXIS2_PLACEMENT_3D('',#47139,#30617,#30618);
#28325=AXIS2_PLACEMENT_3D('',#47301,#30620,#30621);
#28326=AXIS2_PLACEMENT_3D('',#47568,#30623,#30624);
#28327=AXIS2_PLACEMENT_3D('',#47846,#30626,#30627);
#28328=AXIS2_PLACEMENT_3D('',#48179,#30629,#30630);
#28329=AXIS2_PLACEMENT_3D('',#48344,#30632,#30633);
#28330=AXIS2_PLACEMENT_3D('',#48613,#30635,#30636);
#28331=AXIS2_PLACEMENT_3D('',#48894,#30638,#30639);
#28332=AXIS2_PLACEMENT_3D('',#49227,#30641,#30642);
#28333=AXIS2_PLACEMENT_3D('',#49386,#30644,#30645);
#28334=AXIS2_PLACEMENT_3D('',#49656,#30647,#30648);
#28335=AXIS2_PLACEMENT_3D('',#49937,#30650,#30651);
#28336=AXIS2_PLACEMENT_3D('',#50268,#30653,#30654);
#28337=AXIS2_PLACEMENT_3D('',#50431,#30656,#30657);
#28338=AXIS2_PLACEMENT_3D('',#50697,#30659,#30660);
#28339=AXIS2_PLACEMENT_3D('',#50978,#30662,#30663);
#28340=AXIS2_PLACEMENT_3D('',#51311,#30665,#30666);
#28341=AXIS2_PLACEMENT_3D('',#51592,#30668,#30669);
#28342=AXIS2_PLACEMENT_3D('',#51610,#30671,#30672);
#28343=AXIS2_PLACEMENT_3D('',#51677,#30673,#30674);
#28344=AXIS2_PLACEMENT_3D('',#51697,#30676,#30677);
#28345=AXIS2_PLACEMENT_3D('',#51765,#30678,#30679);
#28346=AXIS2_PLACEMENT_3D('',#51916,#30681,#30682);
#28347=AXIS2_PLACEMENT_3D('',#52249,#30684,#30685);
#28348=AXIS2_PLACEMENT_3D('',#52530,#30687,#30688);
#28349=AXIS2_PLACEMENT_3D('',#52866,#30690,#30691);
#28350=AXIS2_PLACEMENT_3D('',#53028,#30693,#30694);
#28351=AXIS2_PLACEMENT_3D('',#53298,#30696,#30697);
#28352=AXIS2_PLACEMENT_3D('',#53573,#30699,#30700);
#28353=AXIS2_PLACEMENT_3D('',#53907,#30702,#30703);
#28354=AXIS2_PLACEMENT_3D('',#54069,#30705,#30706);
#28355=AXIS2_PLACEMENT_3D('',#54336,#30708,#30709);
#28356=AXIS2_PLACEMENT_3D('',#54614,#30711,#30712);
#28357=AXIS2_PLACEMENT_3D('',#54947,#30714,#30715);
#28358=AXIS2_PLACEMENT_3D('',#55112,#30717,#30718);
#28359=AXIS2_PLACEMENT_3D('',#55381,#30720,#30721);
#28360=AXIS2_PLACEMENT_3D('',#55662,#30723,#30724);
#28361=AXIS2_PLACEMENT_3D('',#55995,#30726,#30727);
#28362=AXIS2_PLACEMENT_3D('',#56154,#30729,#30730);
#28363=AXIS2_PLACEMENT_3D('',#56424,#30732,#30733);
#28364=AXIS2_PLACEMENT_3D('',#56705,#30735,#30736);
#28365=AXIS2_PLACEMENT_3D('',#57036,#30738,#30739);
#28366=AXIS2_PLACEMENT_3D('',#57199,#30741,#30742);
#28367=AXIS2_PLACEMENT_3D('',#57465,#30744,#30745);
#28368=AXIS2_PLACEMENT_3D('',#57746,#30747,#30748);
#28369=AXIS2_PLACEMENT_3D('',#58079,#30750,#30751);
#28370=AXIS2_PLACEMENT_3D('',#58360,#30753,#30754);
#28371=AXIS2_PLACEMENT_3D('',#58378,#30756,#30757);
#28372=AXIS2_PLACEMENT_3D('',#58445,#30758,#30759);
#28373=AXIS2_PLACEMENT_3D('',#58465,#30761,#30762);
#28374=AXIS2_PLACEMENT_3D('',#58533,#30763,#30764);
#28375=AXIS2_PLACEMENT_3D('',#58684,#30766,#30767);
#28376=AXIS2_PLACEMENT_3D('',#59017,#30769,#30770);
#28377=AXIS2_PLACEMENT_3D('',#59298,#30772,#30773);
#28378=AXIS2_PLACEMENT_3D('',#59634,#30775,#30776);
#28379=AXIS2_PLACEMENT_3D('',#59796,#30778,#30779);
#28380=AXIS2_PLACEMENT_3D('',#60066,#30781,#30782);
#28381=AXIS2_PLACEMENT_3D('',#60341,#30784,#30785);
#28382=AXIS2_PLACEMENT_3D('',#60675,#30787,#30788);
#28383=AXIS2_PLACEMENT_3D('',#60837,#30790,#30791);
#28384=AXIS2_PLACEMENT_3D('',#61104,#30793,#30794);
#28385=AXIS2_PLACEMENT_3D('',#61382,#30796,#30797);
#28386=AXIS2_PLACEMENT_3D('',#61715,#30799,#30800);
#28387=AXIS2_PLACEMENT_3D('',#61880,#30802,#30803);
#28388=AXIS2_PLACEMENT_3D('',#62149,#30805,#30806);
#28389=AXIS2_PLACEMENT_3D('',#62430,#30808,#30809);
#28390=AXIS2_PLACEMENT_3D('',#62763,#30811,#30812);
#28391=AXIS2_PLACEMENT_3D('',#62922,#30814,#30815);
#28392=AXIS2_PLACEMENT_3D('',#63192,#30817,#30818);
#28393=AXIS2_PLACEMENT_3D('',#63473,#30820,#30821);
#28394=AXIS2_PLACEMENT_3D('',#63804,#30823,#30824);
#28395=AXIS2_PLACEMENT_3D('',#63967,#30826,#30827);
#28396=AXIS2_PLACEMENT_3D('',#64233,#30829,#30830);
#28397=AXIS2_PLACEMENT_3D('',#64514,#30832,#30833);
#28398=AXIS2_PLACEMENT_3D('',#64847,#30835,#30836);
#28399=AXIS2_PLACEMENT_3D('',#65128,#30838,#30839);
#28400=AXIS2_PLACEMENT_3D('',#65146,#30841,#30842);
#28401=AXIS2_PLACEMENT_3D('',#65213,#30843,#30844);
#28402=AXIS2_PLACEMENT_3D('',#65257,#30846,#30847);
#28403=AXIS2_PLACEMENT_3D('',#65290,#30848,#30849);
#28404=AXIS2_PLACEMENT_3D('',#65590,#30851,#30852);
#28405=AXIS2_PLACEMENT_3D('',#66043,#30854,#30855);
#28406=AXIS2_PLACEMENT_3D('',#66048,#30857,#30858);
#28407=AXIS2_PLACEMENT_3D('',#66063,#30859,#30860);
#28408=AXIS2_PLACEMENT_3D('',#66068,#30862,#30863);
#28409=AXIS2_PLACEMENT_3D('',#66083,#30864,#30865);
#28410=AXIS2_PLACEMENT_3D('',#66302,#30867,#30868);
#28411=AXIS2_PLACEMENT_3D('',#66357,#30869,#30870);
#28412=AXIS2_PLACEMENT_3D('',#66810,#30872,#30873);
#28413=AXIS2_PLACEMENT_3D('',#66854,#30875,#30876);
#28414=AXIS2_PLACEMENT_3D('',#66887,#30877,#30878);
#28415=AXIS2_PLACEMENT_3D('',#67038,#30880,#30881);
#28416=AXIS2_PLACEMENT_3D('',#67217,#30882,#30883);
#28417=AXIS2_PLACEMENT_3D('',#67687,#30885,#30886);
#28418=AXIS2_PLACEMENT_3D('',#68143,#30888,#30889);
#28419=AXIS2_PLACEMENT_3D('',#68401,#30891,#30892);
#28420=AXIS2_PLACEMENT_3D('',#68848,#30894,#30895);
#28421=AXIS2_PLACEMENT_3D('',#69358,#30897,#30898);
#28422=AXIS2_PLACEMENT_3D('',#69864,#30900,#30901);
#28423=AXIS2_PLACEMENT_3D('',#70340,#30903,#30904);
#28424=AXIS2_PLACEMENT_3D('',#70824,#30906,#30907);
#28425=AXIS2_PLACEMENT_3D('',#71116,#30909,#30910);
#28426=AXIS2_PLACEMENT_3D('',#71552,#30912,#30913);
#28427=AXIS2_PLACEMENT_3D('',#71963,#30915,#30916);
#28428=AXIS2_PLACEMENT_3D('',#72233,#30918,#30919);
#28429=AXIS2_PLACEMENT_3D('',#72743,#30921,#30922);
#28430=AXIS2_PLACEMENT_3D('',#73246,#30924,#30925);
#28431=AXIS2_PLACEMENT_3D('',#73510,#30927,#30928);
#28432=AXIS2_PLACEMENT_3D('',#73944,#30930,#30931);
#28433=AXIS2_PLACEMENT_3D('',#74367,#30933,#30934);
#28434=AXIS2_PLACEMENT_3D('',#74661,#30936,#30937);
#28435=AXIS2_PLACEMENT_3D('',#75135,#30939,#30940);
#28436=AXIS2_PLACEMENT_3D('',#75621,#30942,#30943);
#28437=AXIS2_PLACEMENT_3D('',#76121,#30945,#30946);
#28438=AXIS2_PLACEMENT_3D('',#76635,#30948,#30949);
#28439=AXIS2_PLACEMENT_3D('',#77055,#30951,#30952);
#28440=AXIS2_PLACEMENT_3D('',#77313,#30954,#30955);
#28441=AXIS2_PLACEMENT_3D('',#77775,#30957,#30958);
#28442=AXIS2_PLACEMENT_3D('',#77887,#30960,#30961);
#28443=AXIS2_PLACEMENT_3D('',#78048,#30962,#30963);
#28444=AXIS2_PLACEMENT_3D('',#78199,#30965,#30966);
#28445=AXIS2_PLACEMENT_3D('',#78378,#30967,#30968);
#28446=AXIS2_PLACEMENT_3D('',#78842,#30970,#30971);
#28447=AXIS2_PLACEMENT_3D('',#79300,#30973,#30974);
#28448=AXIS2_PLACEMENT_3D('',#79556,#30976,#30977);
#28449=AXIS2_PLACEMENT_3D('',#80001,#30979,#30980);
#28450=AXIS2_PLACEMENT_3D('',#80511,#30982,#30983);
#28451=AXIS2_PLACEMENT_3D('',#81015,#30985,#30986);
#28452=AXIS2_PLACEMENT_3D('',#81525,#30988,#30989);
#28453=AXIS2_PLACEMENT_3D('',#81999,#30991,#30992);
#28454=AXIS2_PLACEMENT_3D('',#82291,#30994,#30995);
#28455=AXIS2_PLACEMENT_3D('',#82723,#30997,#30998);
#28456=AXIS2_PLACEMENT_3D('',#83134,#31000,#31001);
#28457=AXIS2_PLACEMENT_3D('',#83408,#31003,#31004);
#28458=AXIS2_PLACEMENT_3D('',#83900,#31006,#31007);
#28459=AXIS2_PLACEMENT_3D('',#84401,#31009,#31010);
#28460=AXIS2_PLACEMENT_3D('',#84657,#31012,#31013);
#28461=AXIS2_PLACEMENT_3D('',#85089,#31015,#31016);
#28462=AXIS2_PLACEMENT_3D('',#85512,#31018,#31019);
#28463=AXIS2_PLACEMENT_3D('',#85808,#31021,#31022);
#28464=AXIS2_PLACEMENT_3D('',#86286,#31024,#31025);
#28465=AXIS2_PLACEMENT_3D('',#86816,#31027,#31028);
#28466=AXIS2_PLACEMENT_3D('',#87312,#31030,#31031);
#28467=AXIS2_PLACEMENT_3D('',#87846,#31033,#31034);
#28468=AXIS2_PLACEMENT_3D('',#88266,#31036,#31037);
#28469=AXIS2_PLACEMENT_3D('',#88526,#31039,#31040);
#28470=AXIS2_PLACEMENT_3D('',#88992,#31042,#31043);
#28471=AXIS2_PLACEMENT_3D('',#89104,#31045,#31046);
#28472=AXIS2_PLACEMENT_3D('',#89265,#31047,#31048);
#28473=AXIS2_PLACEMENT_3D('',#89416,#31050,#31051);
#28474=AXIS2_PLACEMENT_3D('',#89595,#31052,#31053);
#28475=AXIS2_PLACEMENT_3D('',#90057,#31055,#31056);
#28476=AXIS2_PLACEMENT_3D('',#90513,#31058,#31059);
#28477=AXIS2_PLACEMENT_3D('',#90763,#31061,#31062);
#28478=AXIS2_PLACEMENT_3D('',#91208,#31064,#31065);
#28479=AXIS2_PLACEMENT_3D('',#91730,#31067,#31068);
#28480=AXIS2_PLACEMENT_3D('',#92234,#31070,#31071);
#28481=AXIS2_PLACEMENT_3D('',#92700,#31073,#31074);
#28482=AXIS2_PLACEMENT_3D('',#93174,#31076,#31077);
#28483=AXIS2_PLACEMENT_3D('',#93466,#31079,#31080);
#28484=AXIS2_PLACEMENT_3D('',#93898,#31082,#31083);
#28485=AXIS2_PLACEMENT_3D('',#94309,#31085,#31086);
#28486=AXIS2_PLACEMENT_3D('',#94577,#31088,#31089);
#28487=AXIS2_PLACEMENT_3D('',#95071,#31091,#31092);
#28488=AXIS2_PLACEMENT_3D('',#95572,#31094,#31095);
#28489=AXIS2_PLACEMENT_3D('',#95836,#31097,#31098);
#28490=AXIS2_PLACEMENT_3D('',#96270,#31100,#31101);
#28491=AXIS2_PLACEMENT_3D('',#96691,#31103,#31104);
#28492=AXIS2_PLACEMENT_3D('',#96985,#31106,#31107);
#28493=AXIS2_PLACEMENT_3D('',#97463,#31109,#31110);
#28494=AXIS2_PLACEMENT_3D('',#97949,#31112,#31113);
#28495=AXIS2_PLACEMENT_3D('',#98445,#31115,#31116);
#28496=AXIS2_PLACEMENT_3D('',#98959,#31118,#31119);
#28497=AXIS2_PLACEMENT_3D('',#99379,#31121,#31122);
#28498=AXIS2_PLACEMENT_3D('',#99641,#31124,#31125);
#28499=AXIS2_PLACEMENT_3D('',#100103,#31127,#31128);
#28500=AXIS2_PLACEMENT_3D('',#100215,#31130,#31131);
#28501=AXIS2_PLACEMENT_3D('',#100376,#31132,#31133);
#28502=AXIS2_PLACEMENT_3D('',#100527,#31135,#31136);
#28503=AXIS2_PLACEMENT_3D('',#100706,#31137,#31138);
#28504=AXIS2_PLACEMENT_3D('',#101176,#31140,#31141);
#28505=AXIS2_PLACEMENT_3D('',#101634,#31143,#31144);
#28506=AXIS2_PLACEMENT_3D('',#101888,#31146,#31147);
#28507=AXIS2_PLACEMENT_3D('',#102333,#31149,#31150);
#28508=AXIS2_PLACEMENT_3D('',#102841,#31152,#31153);
#28509=AXIS2_PLACEMENT_3D('',#103345,#31155,#31156);
#28510=AXIS2_PLACEMENT_3D('',#103867,#31158,#31159);
#28511=AXIS2_PLACEMENT_3D('',#104351,#31161,#31162);
#28512=AXIS2_PLACEMENT_3D('',#104645,#31164,#31165);
#28513=AXIS2_PLACEMENT_3D('',#105081,#31167,#31168);
#28514=AXIS2_PLACEMENT_3D('',#105492,#31170,#31171);
#28515=AXIS2_PLACEMENT_3D('',#105756,#31173,#31174);
#28516=AXIS2_PLACEMENT_3D('',#106248,#31176,#31177);
#28517=AXIS2_PLACEMENT_3D('',#106801,#31179,#31180);
#28518=AXIS2_PLACEMENT_3D('',#107061,#31182,#31183);
#28519=AXIS2_PLACEMENT_3D('',#107493,#31185,#31186);
#28520=AXIS2_PLACEMENT_3D('',#107916,#31188,#31189);
#28521=AXIS2_PLACEMENT_3D('',#108212,#31191,#31192);
#28522=AXIS2_PLACEMENT_3D('',#108686,#31194,#31195);
#28523=AXIS2_PLACEMENT_3D('',#109164,#31197,#31198);
#28524=AXIS2_PLACEMENT_3D('',#109660,#31200,#31201);
#28525=AXIS2_PLACEMENT_3D('',#110184,#31203,#31204);
#28526=AXIS2_PLACEMENT_3D('',#110604,#31206,#31207);
#28527=AXIS2_PLACEMENT_3D('',#110864,#31209,#31210);
#28528=AXIS2_PLACEMENT_3D('',#111326,#31212,#31213);
#28529=AXIS2_PLACEMENT_3D('',#111438,#31215,#31216);
#28530=AXIS2_PLACEMENT_3D('',#111599,#31217,#31218);
#28531=AXIS2_PLACEMENT_3D('',#112074,#31219,#31220);
#28532=AXIS2_PLACEMENT_3D('',#112551,#31221,#31222);
#28533=AXIS2_PLACEMENT_3D('',#113028,#31223,#31224);
#28534=AXIS2_PLACEMENT_3D('',#113495,#31225,#31226);
#28535=AXIS2_PLACEMENT_3D('',#113790,#31227,#31228);
#28536=AXIS2_PLACEMENT_3D('',#114060,#31229,#31230);
#28537=AXIS2_PLACEMENT_3D('',#114061,#31231,#31232);
#28538=AXIS2_PLACEMENT_3D('',#114156,#31233,#31234);
#28539=AXIS2_PLACEMENT_3D('',#114251,#31235,#31236);
#28540=AXIS2_PLACEMENT_3D('',#114346,#31237,#31238);
#28541=AXIS2_PLACEMENT_3D('',#114441,#31239,#31240);
#28542=AXIS2_PLACEMENT_3D('',#114777,#31241,#31242);
#28543=AXIS2_PLACEMENT_3D('',#115113,#31243,#31244);
#28544=AXIS2_PLACEMENT_3D('',#115115,#31245,#31246);
#28545=AXIS2_PLACEMENT_3D('',#115118,#31248,#31249);
#28546=AXIS2_PLACEMENT_3D('',#115119,#31250,#31251);
#28547=AXIS2_PLACEMENT_3D('',#115120,#31252,#31253);
#28548=AXIS2_PLACEMENT_3D('',#115123,#31254,#31255);
#28549=AXIS2_PLACEMENT_3D('',#115127,#31257,#31258);
#28550=AXIS2_PLACEMENT_3D('',#115129,#31260,#31261);
#28551=AXIS2_PLACEMENT_3D('',#115136,#31265,#31266);
#28552=AXIS2_PLACEMENT_3D('',#115137,#31267,#31268);
#28553=AXIS2_PLACEMENT_3D('',#115139,#31269,#31270);
#28554=AXIS2_PLACEMENT_3D('',#115142,#31272,#31273);
#28555=AXIS2_PLACEMENT_3D('',#115143,#31274,#31275);
#28556=AXIS2_PLACEMENT_3D('',#115144,#31276,#31277);
#28557=AXIS2_PLACEMENT_3D('',#115147,#31278,#31279);
#28558=AXIS2_PLACEMENT_3D('',#115151,#31281,#31282);
#28559=AXIS2_PLACEMENT_3D('',#115153,#31284,#31285);
#28560=AXIS2_PLACEMENT_3D('',#115160,#31289,#31290);
#28561=AXIS2_PLACEMENT_3D('',#115161,#31291,#31292);
#28562=AXIS2_PLACEMENT_3D('',#115163,#31293,#31294);
#28563=AXIS2_PLACEMENT_3D('',#115166,#31296,#31297);
#28564=AXIS2_PLACEMENT_3D('',#115167,#31298,#31299);
#28565=AXIS2_PLACEMENT_3D('',#115168,#31300,#31301);
#28566=AXIS2_PLACEMENT_3D('',#115174,#31305,#31306);
#28567=AXIS2_PLACEMENT_3D('',#115182,#31311,#31312);
#28568=AXIS2_PLACEMENT_3D('',#115187,#31316,#31317);
#28569=AXIS2_PLACEMENT_3D('',#115191,#31319,#31320);
#28570=AXIS2_PLACEMENT_3D('',#115195,#31322,#31323);
#28571=AXIS2_PLACEMENT_3D('',#115199,#31325,#31326);
#28572=AXIS2_PLACEMENT_3D('',#115203,#31328,#31329);
#28573=AXIS2_PLACEMENT_3D('',#115215,#31335,#31336);
#28574=AXIS2_PLACEMENT_3D('',#115219,#31338,#31339);
#28575=AXIS2_PLACEMENT_3D('',#115231,#31345,#31346);
#28576=AXIS2_PLACEMENT_3D('',#115235,#31348,#31349);
#28577=AXIS2_PLACEMENT_3D('',#115239,#31351,#31352);
#28578=AXIS2_PLACEMENT_3D('',#115242,#31354,#31355);
#28579=AXIS2_PLACEMENT_3D('',#115244,#31356,#31357);
#28580=AXIS2_PLACEMENT_3D('',#115246,#31358,#31359);
#28581=AXIS2_PLACEMENT_3D('',#124042,#31360,#31361);
#28582=AXIS2_PLACEMENT_3D('',#124051,#31366,#31367);
#28583=AXIS2_PLACEMENT_3D('',#124057,#31371,#31372);
#28584=AXIS2_PLACEMENT_3D('',#124063,#31376,#31377);
#28585=AXIS2_PLACEMENT_3D('',#124069,#31381,#31382);
#28586=AXIS2_PLACEMENT_3D('',#124075,#31386,#31387);
#28587=AXIS2_PLACEMENT_3D('',#124081,#31391,#31392);
#28588=AXIS2_PLACEMENT_3D('',#124084,#31395,#31396);
#28589=AXIS2_PLACEMENT_3D('',#124086,#31397,#31398);
#28590=AXIS2_PLACEMENT_3D('',#124089,#31400,#31401);
#28591=AXIS2_PLACEMENT_3D('',#124090,#31402,#31403);
#28592=AXIS2_PLACEMENT_3D('',#124091,#31404,#31405);
#28593=AXIS2_PLACEMENT_3D('',#124094,#31406,#31407);
#28594=AXIS2_PLACEMENT_3D('',#124098,#31409,#31410);
#28595=AXIS2_PLACEMENT_3D('',#124100,#31412,#31413);
#28596=AXIS2_PLACEMENT_3D('',#124106,#31417,#31418);
#28597=AXIS2_PLACEMENT_3D('',#124108,#31419,#31420);
#28598=AXIS2_PLACEMENT_3D('',#124110,#31421,#31422);
#28599=AXIS2_PLACEMENT_3D('',#124112,#31424,#31425);
#28600=AXIS2_PLACEMENT_3D('',#124115,#31428,#31429);
#28601=AXIS2_PLACEMENT_3D('',#124118,#31432,#31433);
#28602=AXIS2_PLACEMENT_3D('',#124120,#31434,#31435);
#28603=AXIS2_PLACEMENT_3D('',#124122,#31436,#31437);
#28604=AXIS2_PLACEMENT_3D('',#124123,#31438,#31439);
#28605=AXIS2_PLACEMENT_3D('',#124132,#31444,#31445);
#28606=AXIS2_PLACEMENT_3D('',#124138,#31449,#31450);
#28607=AXIS2_PLACEMENT_3D('',#124144,#31454,#31455);
#28608=AXIS2_PLACEMENT_3D('',#124150,#31459,#31460);
#28609=AXIS2_PLACEMENT_3D('',#124156,#31464,#31465);
#28610=AXIS2_PLACEMENT_3D('',#124162,#31469,#31470);
#28611=AXIS2_PLACEMENT_3D('',#124165,#31473,#31474);
#28612=AXIS2_PLACEMENT_3D('',#124167,#31475,#31476);
#28613=AXIS2_PLACEMENT_3D('',#124170,#31478,#31479);
#28614=AXIS2_PLACEMENT_3D('',#124171,#31480,#31481);
#28615=AXIS2_PLACEMENT_3D('',#124172,#31482,#31483);
#28616=AXIS2_PLACEMENT_3D('',#124173,#31484,#31485);
#28617=AXIS2_PLACEMENT_3D('',#124174,#31486,#31487);
#28618=AXIS2_PLACEMENT_3D('',#124176,#31488,#31489);
#28619=AXIS2_PLACEMENT_3D('',#124178,#31491,#31492);
#28620=AXIS2_PLACEMENT_3D('',#124179,#31493,#31494);
#28621=AXIS2_PLACEMENT_3D('',#124180,#31495,#31496);
#28622=AXIS2_PLACEMENT_3D('',#124182,#31497,#31498);
#28623=AXIS2_PLACEMENT_3D('',#124184,#31500,#31501);
#28624=AXIS2_PLACEMENT_3D('',#124185,#31502,#31503);
#28625=AXIS2_PLACEMENT_3D('',#124188,#31504,#31505);
#28626=AXIS2_PLACEMENT_3D('',#124192,#31507,#31508);
#28627=AXIS2_PLACEMENT_3D('',#124194,#31510,#31511);
#28628=AXIS2_PLACEMENT_3D('',#124200,#31515,#31516);
#28629=AXIS2_PLACEMENT_3D('',#124202,#31517,#31518);
#28630=AXIS2_PLACEMENT_3D('',#124205,#31520,#31521);
#28631=AXIS2_PLACEMENT_3D('',#124206,#31522,#31523);
#28632=AXIS2_PLACEMENT_3D('',#124209,#31526,#31527);
#28633=AXIS2_PLACEMENT_3D('',#124212,#31530,#31531);
#28634=AXIS2_PLACEMENT_3D('',#124214,#31532,#31533);
#28635=AXIS2_PLACEMENT_3D('',#124216,#31534,#31535);
#28636=AXIS2_PLACEMENT_3D('',#124217,#31536,#31537);
#28637=AXIS2_PLACEMENT_3D('',#124226,#31542,#31543);
#28638=AXIS2_PLACEMENT_3D('',#124232,#31547,#31548);
#28639=AXIS2_PLACEMENT_3D('',#124238,#31552,#31553);
#28640=AXIS2_PLACEMENT_3D('',#124244,#31557,#31558);
#28641=AXIS2_PLACEMENT_3D('',#124250,#31562,#31563);
#28642=AXIS2_PLACEMENT_3D('',#124256,#31567,#31568);
#28643=AXIS2_PLACEMENT_3D('',#124259,#31571,#31572);
#28644=AXIS2_PLACEMENT_3D('',#124261,#31573,#31574);
#28645=AXIS2_PLACEMENT_3D('',#124264,#31576,#31577);
#28646=AXIS2_PLACEMENT_3D('',#124265,#31578,#31579);
#28647=AXIS2_PLACEMENT_3D('',#124266,#31580,#31581);
#28648=AXIS2_PLACEMENT_3D('',#124275,#31586,#31587);
#28649=AXIS2_PLACEMENT_3D('',#124281,#31591,#31592);
#28650=AXIS2_PLACEMENT_3D('',#124287,#31596,#31597);
#28651=AXIS2_PLACEMENT_3D('',#124293,#31601,#31602);
#28652=AXIS2_PLACEMENT_3D('',#124299,#31606,#31607);
#28653=AXIS2_PLACEMENT_3D('',#124305,#31611,#31612);
#28654=AXIS2_PLACEMENT_3D('',#124308,#31615,#31616);
#28655=AXIS2_PLACEMENT_3D('',#124310,#31617,#31618);
#28656=AXIS2_PLACEMENT_3D('',#124313,#31620,#31621);
#28657=AXIS2_PLACEMENT_3D('',#124314,#31622,#31623);
#28658=AXIS2_PLACEMENT_3D('',#124315,#31624,#31625);
#28659=AXIS2_PLACEMENT_3D('',#124316,#31626,#31627);
#28660=AXIS2_PLACEMENT_3D('',#124317,#31628,#31629);
#28661=AXIS2_PLACEMENT_3D('',#124323,#31633,#31634);
#28662=AXIS2_PLACEMENT_3D('',#124324,#31635,#31636);
#28663=AXIS2_PLACEMENT_3D('',#124327,#31638,#31639);
#28664=AXIS2_PLACEMENT_3D('',#124328,#31640,#31641);
#28665=AXIS2_PLACEMENT_3D('',#124329,#31642,#31643);
#28666=AXIS2_PLACEMENT_3D('',#124332,#31645,#31646);
#28667=AXIS2_PLACEMENT_3D('',#124333,#31647,#31648);
#28668=AXIS2_PLACEMENT_3D('',#124334,#31649,#31650);
#28669=AXIS2_PLACEMENT_3D('',#124337,#31652,#31653);
#28670=AXIS2_PLACEMENT_3D('',#124338,#31654,#31655);
#28671=AXIS2_PLACEMENT_3D('',#124339,#31656,#31657);
#28672=AXIS2_PLACEMENT_3D('',#124342,#31659,#31660);
#28673=AXIS2_PLACEMENT_3D('',#124343,#31661,#31662);
#28674=AXIS2_PLACEMENT_3D('',#124344,#31663,#31664);
#28675=AXIS2_PLACEMENT_3D('',#124348,#31667,#31668);
#28676=AXIS2_PLACEMENT_3D('',#124349,#31669,#31670);
#28677=AXIS2_PLACEMENT_3D('',#124350,#31671,#31672);
#28678=AXIS2_PLACEMENT_3D('',#124352,#31673,#31674);
#28679=AXIS2_PLACEMENT_3D('',#124354,#31676,#31677);
#28680=AXIS2_PLACEMENT_3D('',#124358,#31680,#31681);
#28681=AXIS2_PLACEMENT_3D('',#124360,#31682,#31683);
#28682=AXIS2_PLACEMENT_3D('',#124362,#31685,#31686);
#28683=AXIS2_PLACEMENT_3D('',#124366,#31689,#31690);
#28684=AXIS2_PLACEMENT_3D('',#124368,#31691,#31692);
#28685=AXIS2_PLACEMENT_3D('',#124370,#31694,#31695);
#28686=AXIS2_PLACEMENT_3D('',#124374,#31698,#31699);
#28687=AXIS2_PLACEMENT_3D('',#124375,#31700,#31701);
#28688=AXIS2_PLACEMENT_3D('',#124376,#31702,#31703);
#28689=AXIS2_PLACEMENT_3D('',#124378,#31704,#31705);
#28690=AXIS2_PLACEMENT_3D('',#124380,#31707,#31708);
#28691=AXIS2_PLACEMENT_3D('',#124384,#31711,#31712);
#28692=AXIS2_PLACEMENT_3D('',#124386,#31713,#31714);
#28693=AXIS2_PLACEMENT_3D('',#124388,#31716,#31717);
#28694=AXIS2_PLACEMENT_3D('',#124392,#31720,#31721);
#28695=AXIS2_PLACEMENT_3D('',#124394,#31722,#31723);
#28696=AXIS2_PLACEMENT_3D('',#124396,#31725,#31726);
#28697=AXIS2_PLACEMENT_3D('',#124400,#31729,#31730);
#28698=AXIS2_PLACEMENT_3D('',#124402,#31731,#31732);
#28699=AXIS2_PLACEMENT_3D('',#124404,#31734,#31735);
#28700=AXIS2_PLACEMENT_3D('',#124408,#31738,#31739);
#28701=AXIS2_PLACEMENT_3D('',#124410,#31740,#31741);
#28702=AXIS2_PLACEMENT_3D('',#124412,#31743,#31744);
#28703=AXIS2_PLACEMENT_3D('',#124416,#31747,#31748);
#28704=AXIS2_PLACEMENT_3D('',#124418,#31749,#31750);
#28705=AXIS2_PLACEMENT_3D('',#124420,#31752,#31753);
#28706=AXIS2_PLACEMENT_3D('',#124424,#31756,#31757);
#28707=AXIS2_PLACEMENT_3D('',#124425,#31758,#31759);
#28708=AXIS2_PLACEMENT_3D('',#124426,#31760,#31761);
#30469=DIRECTION('axis',(0.,0.,1.));
#30470=DIRECTION('refdir',(1.,0.,0.));
#30471=DIRECTION('center_axis',(1.,0.,0.));
#30472=DIRECTION('ref_axis',(0.,-0.793547993282919,-0.608507668280895));
#30473=DIRECTION('',(1.,0.,0.));
#30474=DIRECTION('center_axis',(-1.,0.,0.));
#30475=DIRECTION('ref_axis',(0.,-1.74186785585433E-15,1.));
#30476=DIRECTION('center_axis',(1.,0.,0.));
#30477=DIRECTION('ref_axis',(0.,-0.793547993282919,-0.608507668280895));
#30478=DIRECTION('',(1.,0.,0.));
#30479=DIRECTION('center_axis',(1.,0.,0.));
#30480=DIRECTION('ref_axis',(0.,-0.793547993282919,-0.608507668280895));
#30481=DIRECTION('',(1.,0.,0.));
#30482=DIRECTION('center_axis',(1.,0.,0.));
#30483=DIRECTION('ref_axis',(0.,-0.793547993282919,-0.608507668280895));
#30484=DIRECTION('',(1.,0.,0.));
#30485=DIRECTION('center_axis',(1.,0.,0.));
#30486=DIRECTION('ref_axis',(0.,-1.74186785585433E-15,1.));
#30487=DIRECTION('center_axis',(-1.,0.,0.));
#30488=DIRECTION('ref_axis',(0.,0.793547993033681,-0.608507668605924));
#30489=DIRECTION('',(-1.,0.,0.));
#30490=DIRECTION('center_axis',(1.,0.,0.));
#30491=DIRECTION('ref_axis',(0.,-1.74186785585433E-15,1.));
#30492=DIRECTION('center_axis',(-1.,0.,0.));
#30493=DIRECTION('ref_axis',(0.,0.793547993033681,-0.608507668605924));
#30494=DIRECTION('',(-1.,0.,0.));
#30495=DIRECTION('center_axis',(-1.,0.,0.));
#30496=DIRECTION('ref_axis',(0.,0.793547993033681,-0.608507668605924));
#30497=DIRECTION('',(-1.,0.,0.));
#30498=DIRECTION('center_axis',(-1.,0.,0.));
#30499=DIRECTION('ref_axis',(0.,0.793547993033681,-0.608507668605924));
#30500=DIRECTION('',(-1.,0.,0.));
#30501=DIRECTION('center_axis',(-1.,0.,0.));
#30502=DIRECTION('ref_axis',(0.,-1.74186785585433E-15,1.));
#30503=DIRECTION('center_axis',(0.,0.,-1.));
#30504=DIRECTION('ref_axis',(-0.609193654691519,-0.793021494717256,0.));
#30505=DIRECTION('',(0.,0.,-1.));
#30506=DIRECTION('center_axis',(0.,0.,1.));
#30507=DIRECTION('ref_axis',(1.,8.06646416329218E-14,0.));
#30508=DIRECTION('center_axis',(0.,0.,-1.));
#30509=DIRECTION('ref_axis',(-0.609193654691519,-0.793021494717256,0.));
#30510=DIRECTION('',(0.,0.,-1.));
#30511=DIRECTION('center_axis',(0.,0.,-1.));
#30512=DIRECTION('ref_axis',(-0.609193654691519,-0.793021494717256,0.));
#30513=DIRECTION('',(0.,0.,-1.));
#30514=DIRECTION('center_axis',(0.,0.,-1.));
#30515=DIRECTION('ref_axis',(-0.609193654691519,-0.793021494717256,0.));
#30516=DIRECTION('',(0.,0.,-1.));
#30517=DIRECTION('center_axis',(0.,0.,-1.));
#30518=DIRECTION('ref_axis',(-0.609193654691519,-0.793021494717256,0.));
#30519=DIRECTION('',(0.,0.,-1.));
#30520=DIRECTION('center_axis',(0.,0.,-1.));
#30521=DIRECTION('ref_axis',(-0.609193654691519,-0.793021494717256,0.));
#30522=DIRECTION('',(0.,0.,-1.));
#30523=DIRECTION('center_axis',(0.,0.,-1.));
#30524=DIRECTION('ref_axis',(-0.609193654691519,-0.793021494717256,0.));
#30525=DIRECTION('',(0.,0.,-1.));
#30526=DIRECTION('center_axis',(0.,0.,-1.));
#30527=DIRECTION('ref_axis',(-0.609193654691519,-0.793021494717256,0.));
#30528=DIRECTION('',(0.,0.,-1.));
#30529=DIRECTION('center_axis',(0.,0.,-1.));
#30530=DIRECTION('ref_axis',(-0.609193654691519,-0.793021494717256,0.));
#30531=DIRECTION('',(0.,0.,-1.));
#30532=DIRECTION('center_axis',(0.,0.,-1.));
#30533=DIRECTION('ref_axis',(-0.609193654691519,-0.793021494717256,0.));
#30534=DIRECTION('',(0.,0.,-1.));
#30535=DIRECTION('center_axis',(0.,0.,-1.));
#30536=DIRECTION('ref_axis',(-0.609193654691519,-0.793021494717256,0.));
#30537=DIRECTION('',(0.,0.,-1.));
#30538=DIRECTION('center_axis',(0.,0.,-1.));
#30539=DIRECTION('ref_axis',(-0.609193654691519,-0.793021494717256,0.));
#30540=DIRECTION('',(0.,0.,-1.));
#30541=DIRECTION('center_axis',(0.,0.,-1.));
#30542=DIRECTION('ref_axis',(-0.609193654691519,-0.793021494717256,0.));
#30543=DIRECTION('',(0.,0.,-1.));
#30544=DIRECTION('center_axis',(0.,0.,-1.));
#30545=DIRECTION('ref_axis',(-0.609193654691519,-0.793021494717256,0.));
#30546=DIRECTION('',(0.,0.,-1.));
#30547=DIRECTION('center_axis',(0.,0.,-1.));
#30548=DIRECTION('ref_axis',(-0.609193654691519,-0.793021494717256,0.));
#30549=DIRECTION('',(0.,0.,-1.));
#30550=DIRECTION('center_axis',(0.,0.,-1.));
#30551=DIRECTION('ref_axis',(-0.609193654691519,-0.793021494717256,0.));
#30552=DIRECTION('',(0.,0.,-1.));
#30553=DIRECTION('center_axis',(0.,0.,-1.));
#30554=DIRECTION('ref_axis',(-0.609193654691519,-0.793021494717256,0.));
#30555=DIRECTION('',(0.,0.,-1.));
#30556=DIRECTION('center_axis',(0.,0.,-1.));
#30557=DIRECTION('ref_axis',(-0.609193654691519,-0.793021494717256,0.));
#30558=DIRECTION('',(0.,0.,-1.));
#30559=DIRECTION('center_axis',(0.,0.,-1.));
#30560=DIRECTION('ref_axis',(-0.609193654691519,-0.793021494717256,0.));
#30561=DIRECTION('',(0.,0.,-1.));
#30562=DIRECTION('center_axis',(0.,0.,-1.));
#30563=DIRECTION('ref_axis',(-0.609193654691519,-0.793021494717256,0.));
#30564=DIRECTION('',(0.,0.,-1.));
#30565=DIRECTION('center_axis',(0.,0.,-1.));
#30566=DIRECTION('ref_axis',(-0.609193654691519,-0.793021494717256,0.));
#30567=DIRECTION('',(0.,0.,-1.));
#30568=DIRECTION('center_axis',(0.,0.,-1.));
#30569=DIRECTION('ref_axis',(-0.609193654691519,-0.793021494717256,0.));
#30570=DIRECTION('',(0.,0.,-1.));
#30571=DIRECTION('center_axis',(0.,0.,-1.));
#30572=DIRECTION('ref_axis',(-0.609193654691519,-0.793021494717256,0.));
#30573=DIRECTION('',(0.,0.,-1.));
#30574=DIRECTION('center_axis',(0.,0.,-1.));
#30575=DIRECTION('ref_axis',(-0.609193654691519,-0.793021494717256,0.));
#30576=DIRECTION('',(0.,0.,-1.));
#30577=DIRECTION('center_axis',(0.,0.,-1.));
#30578=DIRECTION('ref_axis',(-0.609193654691519,-0.793021494717256,0.));
#30579=DIRECTION('',(0.,0.,-1.));
#30580=DIRECTION('center_axis',(0.,0.,-1.));
#30581=DIRECTION('ref_axis',(-0.609193654691519,-0.793021494717256,0.));
#30582=DIRECTION('',(0.,0.,-1.));
#30583=DIRECTION('center_axis',(0.,0.,-1.));
#30584=DIRECTION('ref_axis',(-0.609193654691519,-0.793021494717256,0.));
#30585=DIRECTION('',(0.,0.,-1.));
#30586=DIRECTION('center_axis',(0.,0.,-1.));
#30587=DIRECTION('ref_axis',(1.,8.06646416329218E-14,0.));
#30588=DIRECTION('center_axis',(0.,0.,-1.));
#30589=DIRECTION('ref_axis',(-0.609193705300279,-0.793021455839952,0.));
#30590=DIRECTION('',(0.,0.,-1.));
#30591=DIRECTION('center_axis',(0.,0.,1.));
#30592=DIRECTION('ref_axis',(1.,8.15320033709099E-14,0.));
#30593=DIRECTION('center_axis',(0.,0.,-1.));
#30594=DIRECTION('ref_axis',(-0.609193705300279,-0.793021455839952,0.));
#30595=DIRECTION('',(0.,0.,-1.));
#30596=DIRECTION('center_axis',(0.,0.,-1.));
#30597=DIRECTION('ref_axis',(-0.609193705300279,-0.793021455839952,0.));
#30598=DIRECTION('',(0.,0.,-1.));
#30599=DIRECTION('center_axis',(0.,0.,-1.));
#30600=DIRECTION('ref_axis',(-0.609193705300279,-0.793021455839952,0.));
#30601=DIRECTION('',(0.,0.,-1.));
#30602=DIRECTION('center_axis',(0.,0.,-1.));
#30603=DIRECTION('ref_axis',(-0.609193705300279,-0.793021455839952,0.));
#30604=DIRECTION('',(0.,0.,-1.));
#30605=DIRECTION('center_axis',(0.,0.,-1.));
#30606=DIRECTION('ref_axis',(-0.609193705300279,-0.793021455839952,0.));
#30607=DIRECTION('',(0.,0.,-1.));
#30608=DIRECTION('center_axis',(0.,0.,-1.));
#30609=DIRECTION('ref_axis',(-0.609193705300279,-0.793021455839952,0.));
#30610=DIRECTION('',(0.,0.,-1.));
#30611=DIRECTION('center_axis',(0.,0.,-1.));
#30612=DIRECTION('ref_axis',(-0.609193705300279,-0.793021455839952,0.));
#30613=DIRECTION('',(0.,0.,-1.));
#30614=DIRECTION('center_axis',(0.,0.,-1.));
#30615=DIRECTION('ref_axis',(-0.609193705300279,-0.793021455839952,0.));
#30616=DIRECTION('',(0.,0.,-1.));
#30617=DIRECTION('center_axis',(0.,0.,-1.));
#30618=DIRECTION('ref_axis',(-0.609193705300279,-0.793021455839952,0.));
#30619=DIRECTION('',(0.,0.,-1.));
#30620=DIRECTION('center_axis',(0.,0.,-1.));
#30621=DIRECTION('ref_axis',(-0.609193705300279,-0.793021455839952,0.));
#30622=DIRECTION('',(0.,0.,-1.));
#30623=DIRECTION('center_axis',(0.,0.,-1.));
#30624=DIRECTION('ref_axis',(-0.609193705300279,-0.793021455839952,0.));
#30625=DIRECTION('',(0.,0.,-1.));
#30626=DIRECTION('center_axis',(0.,0.,-1.));
#30627=DIRECTION('ref_axis',(-0.609193705300279,-0.793021455839952,0.));
#30628=DIRECTION('',(0.,0.,-1.));
#30629=DIRECTION('center_axis',(0.,0.,-1.));
#30630=DIRECTION('ref_axis',(-0.609193705300279,-0.793021455839952,0.));
#30631=DIRECTION('',(0.,0.,-1.));
#30632=DIRECTION('center_axis',(0.,0.,-1.));
#30633=DIRECTION('ref_axis',(-0.609193705300279,-0.793021455839952,0.));
#30634=DIRECTION('',(0.,0.,-1.));
#30635=DIRECTION('center_axis',(0.,0.,-1.));
#30636=DIRECTION('ref_axis',(-0.609193705300279,-0.793021455839952,0.));
#30637=DIRECTION('',(0.,0.,-1.));
#30638=DIRECTION('center_axis',(0.,0.,-1.));
#30639=DIRECTION('ref_axis',(-0.609193705300279,-0.793021455839952,0.));
#30640=DIRECTION('',(0.,0.,-1.));
#30641=DIRECTION('center_axis',(0.,0.,-1.));
#30642=DIRECTION('ref_axis',(-0.609193705300279,-0.793021455839952,0.));
#30643=DIRECTION('',(0.,0.,-1.));
#30644=DIRECTION('center_axis',(0.,0.,-1.));
#30645=DIRECTION('ref_axis',(-0.609193705300279,-0.793021455839952,0.));
#30646=DIRECTION('',(0.,0.,-1.));
#30647=DIRECTION('center_axis',(0.,0.,-1.));
#30648=DIRECTION('ref_axis',(-0.609193705300279,-0.793021455839952,0.));
#30649=DIRECTION('',(0.,0.,-1.));
#30650=DIRECTION('center_axis',(0.,0.,-1.));
#30651=DIRECTION('ref_axis',(-0.609193705300279,-0.793021455839952,0.));
#30652=DIRECTION('',(0.,0.,-1.));
#30653=DIRECTION('center_axis',(0.,0.,-1.));
#30654=DIRECTION('ref_axis',(-0.609193705300279,-0.793021455839952,0.));
#30655=DIRECTION('',(0.,0.,-1.));
#30656=DIRECTION('center_axis',(0.,0.,-1.));
#30657=DIRECTION('ref_axis',(-0.609193705300279,-0.793021455839952,0.));
#30658=DIRECTION('',(0.,0.,-1.));
#30659=DIRECTION('center_axis',(0.,0.,-1.));
#30660=DIRECTION('ref_axis',(-0.609193705300279,-0.793021455839952,0.));
#30661=DIRECTION('',(0.,0.,-1.));
#30662=DIRECTION('center_axis',(0.,0.,-1.));
#30663=DIRECTION('ref_axis',(-0.609193705300279,-0.793021455839952,0.));
#30664=DIRECTION('',(0.,0.,-1.));
#30665=DIRECTION('center_axis',(0.,0.,-1.));
#30666=DIRECTION('ref_axis',(-0.609193705300279,-0.793021455839952,0.));
#30667=DIRECTION('',(0.,0.,-1.));
#30668=DIRECTION('center_axis',(0.,0.,-1.));
#30669=DIRECTION('ref_axis',(-0.609193705300279,-0.793021455839952,0.));
#30670=DIRECTION('',(0.,0.,-1.));
#30671=DIRECTION('center_axis',(0.,0.,-1.));
#30672=DIRECTION('ref_axis',(1.,8.15320033709099E-14,0.));
#30673=DIRECTION('center_axis',(0.,0.,-1.));
#30674=DIRECTION('ref_axis',(-0.609193706391024,-0.793021455002049,0.));
#30675=DIRECTION('',(0.,0.,-1.));
#30676=DIRECTION('center_axis',(0.,0.,1.));
#30677=DIRECTION('ref_axis',(1.,7.80625564189562E-14,0.));
#30678=DIRECTION('center_axis',(0.,0.,-1.));
#30679=DIRECTION('ref_axis',(-0.609193706391024,-0.793021455002049,0.));
#30680=DIRECTION('',(0.,0.,-1.));
#30681=DIRECTION('center_axis',(0.,0.,-1.));
#30682=DIRECTION('ref_axis',(-0.609193706391024,-0.793021455002049,0.));
#30683=DIRECTION('',(0.,0.,-1.));
#30684=DIRECTION('center_axis',(0.,0.,-1.));
#30685=DIRECTION('ref_axis',(-0.609193706391024,-0.793021455002049,0.));
#30686=DIRECTION('',(0.,0.,-1.));
#30687=DIRECTION('center_axis',(0.,0.,-1.));
#30688=DIRECTION('ref_axis',(-0.609193706391024,-0.793021455002049,0.));
#30689=DIRECTION('',(0.,0.,-1.));
#30690=DIRECTION('center_axis',(0.,0.,-1.));
#30691=DIRECTION('ref_axis',(-0.609193706391024,-0.793021455002049,0.));
#30692=DIRECTION('',(0.,0.,-1.));
#30693=DIRECTION('center_axis',(0.,0.,-1.));
#30694=DIRECTION('ref_axis',(-0.609193706391024,-0.793021455002049,0.));
#30695=DIRECTION('',(0.,0.,-1.));
#30696=DIRECTION('center_axis',(0.,0.,-1.));
#30697=DIRECTION('ref_axis',(-0.609193706391024,-0.793021455002049,0.));
#30698=DIRECTION('',(0.,0.,-1.));
#30699=DIRECTION('center_axis',(0.,0.,-1.));
#30700=DIRECTION('ref_axis',(-0.609193706391024,-0.793021455002049,0.));
#30701=DIRECTION('',(0.,0.,-1.));
#30702=DIRECTION('center_axis',(0.,0.,-1.));
#30703=DIRECTION('ref_axis',(-0.609193706391024,-0.793021455002049,0.));
#30704=DIRECTION('',(0.,0.,-1.));
#30705=DIRECTION('center_axis',(0.,0.,-1.));
#30706=DIRECTION('ref_axis',(-0.609193706391024,-0.793021455002049,0.));
#30707=DIRECTION('',(0.,0.,-1.));
#30708=DIRECTION('center_axis',(0.,0.,-1.));
#30709=DIRECTION('ref_axis',(-0.609193706391024,-0.793021455002049,0.));
#30710=DIRECTION('',(0.,0.,-1.));
#30711=DIRECTION('center_axis',(0.,0.,-1.));
#30712=DIRECTION('ref_axis',(-0.609193706391024,-0.793021455002049,0.));
#30713=DIRECTION('',(0.,0.,-1.));
#30714=DIRECTION('center_axis',(0.,0.,-1.));
#30715=DIRECTION('ref_axis',(-0.609193706391024,-0.793021455002049,0.));
#30716=DIRECTION('',(0.,0.,-1.));
#30717=DIRECTION('center_axis',(0.,0.,-1.));
#30718=DIRECTION('ref_axis',(-0.609193706391024,-0.793021455002049,0.));
#30719=DIRECTION('',(0.,0.,-1.));
#30720=DIRECTION('center_axis',(0.,0.,-1.));
#30721=DIRECTION('ref_axis',(-0.609193706391024,-0.793021455002049,0.));
#30722=DIRECTION('',(0.,0.,-1.));
#30723=DIRECTION('center_axis',(0.,0.,-1.));
#30724=DIRECTION('ref_axis',(-0.609193706391024,-0.793021455002049,0.));
#30725=DIRECTION('',(0.,0.,-1.));
#30726=DIRECTION('center_axis',(0.,0.,-1.));
#30727=DIRECTION('ref_axis',(-0.609193706391024,-0.793021455002049,0.));
#30728=DIRECTION('',(0.,0.,-1.));
#30729=DIRECTION('center_axis',(0.,0.,-1.));
#30730=DIRECTION('ref_axis',(-0.609193706391024,-0.793021455002049,0.));
#30731=DIRECTION('',(0.,0.,-1.));
#30732=DIRECTION('center_axis',(0.,0.,-1.));
#30733=DIRECTION('ref_axis',(-0.609193706391024,-0.793021455002049,0.));
#30734=DIRECTION('',(0.,0.,-1.));
#30735=DIRECTION('center_axis',(0.,0.,-1.));
#30736=DIRECTION('ref_axis',(-0.609193706391024,-0.793021455002049,0.));
#30737=DIRECTION('',(0.,0.,-1.));
#30738=DIRECTION('center_axis',(0.,0.,-1.));
#30739=DIRECTION('ref_axis',(-0.609193706391024,-0.793021455002049,0.));
#30740=DIRECTION('',(0.,0.,-1.));
#30741=DIRECTION('center_axis',(0.,0.,-1.));
#30742=DIRECTION('ref_axis',(-0.609193706391024,-0.793021455002049,0.));
#30743=DIRECTION('',(0.,0.,-1.));
#30744=DIRECTION('center_axis',(0.,0.,-1.));
#30745=DIRECTION('ref_axis',(-0.609193706391024,-0.793021455002049,0.));
#30746=DIRECTION('',(0.,0.,-1.));
#30747=DIRECTION('center_axis',(0.,0.,-1.));
#30748=DIRECTION('ref_axis',(-0.609193706391024,-0.793021455002049,0.));
#30749=DIRECTION('',(0.,0.,-1.));
#30750=DIRECTION('center_axis',(0.,0.,-1.));
#30751=DIRECTION('ref_axis',(-0.609193706391024,-0.793021455002049,0.));
#30752=DIRECTION('',(0.,0.,-1.));
#30753=DIRECTION('center_axis',(0.,0.,-1.));
#30754=DIRECTION('ref_axis',(-0.609193706391024,-0.793021455002049,0.));
#30755=DIRECTION('',(0.,0.,-1.));
#30756=DIRECTION('center_axis',(0.,0.,-1.));
#30757=DIRECTION('ref_axis',(1.,7.80625564189563E-14,0.));
#30758=DIRECTION('center_axis',(0.,0.,-1.));
#30759=DIRECTION('ref_axis',(-0.60919368949553,-0.793021467981053,0.));
#30760=DIRECTION('',(0.,0.,-1.));
#30761=DIRECTION('center_axis',(0.,0.,1.));
#30762=DIRECTION('ref_axis',(1.,7.89299181569448E-14,0.));
#30763=DIRECTION('center_axis',(0.,0.,-1.));
#30764=DIRECTION('ref_axis',(-0.60919368949553,-0.793021467981053,0.));
#30765=DIRECTION('',(0.,0.,-1.));
#30766=DIRECTION('center_axis',(0.,0.,-1.));
#30767=DIRECTION('ref_axis',(-0.60919368949553,-0.793021467981053,0.));
#30768=DIRECTION('',(0.,0.,-1.));
#30769=DIRECTION('center_axis',(0.,0.,-1.));
#30770=DIRECTION('ref_axis',(-0.60919368949553,-0.793021467981053,0.));
#30771=DIRECTION('',(0.,0.,-1.));
#30772=DIRECTION('center_axis',(0.,0.,-1.));
#30773=DIRECTION('ref_axis',(-0.60919368949553,-0.793021467981053,0.));
#30774=DIRECTION('',(0.,0.,-1.));
#30775=DIRECTION('center_axis',(0.,0.,-1.));
#30776=DIRECTION('ref_axis',(-0.60919368949553,-0.793021467981053,0.));
#30777=DIRECTION('',(0.,0.,-1.));
#30778=DIRECTION('center_axis',(0.,0.,-1.));
#30779=DIRECTION('ref_axis',(-0.60919368949553,-0.793021467981053,0.));
#30780=DIRECTION('',(0.,0.,-1.));
#30781=DIRECTION('center_axis',(0.,0.,-1.));
#30782=DIRECTION('ref_axis',(-0.60919368949553,-0.793021467981053,0.));
#30783=DIRECTION('',(0.,0.,-1.));
#30784=DIRECTION('center_axis',(0.,0.,-1.));
#30785=DIRECTION('ref_axis',(-0.60919368949553,-0.793021467981053,0.));
#30786=DIRECTION('',(0.,0.,-1.));
#30787=DIRECTION('center_axis',(0.,0.,-1.));
#30788=DIRECTION('ref_axis',(-0.60919368949553,-0.793021467981053,0.));
#30789=DIRECTION('',(0.,0.,-1.));
#30790=DIRECTION('center_axis',(0.,0.,-1.));
#30791=DIRECTION('ref_axis',(-0.60919368949553,-0.793021467981053,0.));
#30792=DIRECTION('',(0.,0.,-1.));
#30793=DIRECTION('center_axis',(0.,0.,-1.));
#30794=DIRECTION('ref_axis',(-0.60919368949553,-0.793021467981053,0.));
#30795=DIRECTION('',(0.,0.,-1.));
#30796=DIRECTION('center_axis',(0.,0.,-1.));
#30797=DIRECTION('ref_axis',(-0.60919368949553,-0.793021467981053,0.));
#30798=DIRECTION('',(0.,0.,-1.));
#30799=DIRECTION('center_axis',(0.,0.,-1.));
#30800=DIRECTION('ref_axis',(-0.60919368949553,-0.793021467981053,0.));
#30801=DIRECTION('',(0.,0.,-1.));
#30802=DIRECTION('center_axis',(0.,0.,-1.));
#30803=DIRECTION('ref_axis',(-0.60919368949553,-0.793021467981053,0.));
#30804=DIRECTION('',(0.,0.,-1.));
#30805=DIRECTION('center_axis',(0.,0.,-1.));
#30806=DIRECTION('ref_axis',(-0.60919368949553,-0.793021467981053,0.));
#30807=DIRECTION('',(0.,0.,-1.));
#30808=DIRECTION('center_axis',(0.,0.,-1.));
#30809=DIRECTION('ref_axis',(-0.60919368949553,-0.793021467981053,0.));
#30810=DIRECTION('',(0.,0.,-1.));
#30811=DIRECTION('center_axis',(0.,0.,-1.));
#30812=DIRECTION('ref_axis',(-0.60919368949553,-0.793021467981053,0.));
#30813=DIRECTION('',(0.,0.,-1.));
#30814=DIRECTION('center_axis',(0.,0.,-1.));
#30815=DIRECTION('ref_axis',(-0.60919368949553,-0.793021467981053,0.));
#30816=DIRECTION('',(0.,0.,-1.));
#30817=DIRECTION('center_axis',(0.,0.,-1.));
#30818=DIRECTION('ref_axis',(-0.60919368949553,-0.793021467981053,0.));
#30819=DIRECTION('',(0.,0.,-1.));
#30820=DIRECTION('center_axis',(0.,0.,-1.));
#30821=DIRECTION('ref_axis',(-0.60919368949553,-0.793021467981053,0.));
#30822=DIRECTION('',(0.,0.,-1.));
#30823=DIRECTION('center_axis',(0.,0.,-1.));
#30824=DIRECTION('ref_axis',(-0.60919368949553,-0.793021467981053,0.));
#30825=DIRECTION('',(0.,0.,-1.));
#30826=DIRECTION('center_axis',(0.,0.,-1.));
#30827=DIRECTION('ref_axis',(-0.60919368949553,-0.793021467981053,0.));
#30828=DIRECTION('',(0.,0.,-1.));
#30829=DIRECTION('center_axis',(0.,0.,-1.));
#30830=DIRECTION('ref_axis',(-0.60919368949553,-0.793021467981053,0.));
#30831=DIRECTION('',(0.,0.,-1.));
#30832=DIRECTION('center_axis',(0.,0.,-1.));
#30833=DIRECTION('ref_axis',(-0.60919368949553,-0.793021467981053,0.));
#30834=DIRECTION('',(0.,0.,-1.));
#30835=DIRECTION('center_axis',(0.,0.,-1.));
#30836=DIRECTION('ref_axis',(-0.60919368949553,-0.793021467981053,0.));
#30837=DIRECTION('',(0.,0.,-1.));
#30838=DIRECTION('center_axis',(0.,0.,-1.));
#30839=DIRECTION('ref_axis',(-0.60919368949553,-0.793021467981053,0.));
#30840=DIRECTION('',(0.,0.,-1.));
#30841=DIRECTION('center_axis',(0.,0.,-1.));
#30842=DIRECTION('ref_axis',(1.,7.89299181569448E-14,0.));
#30843=DIRECTION('center_axis',(1.,0.,0.));
#30844=DIRECTION('ref_axis',(0.,0.509892606676753,0.860238065686695));
#30845=DIRECTION('',(1.,0.,0.));
#30846=DIRECTION('center_axis',(-1.,0.,0.));
#30847=DIRECTION('ref_axis',(0.,0.,1.));
#30848=DIRECTION('center_axis',(1.,0.,0.));
#30849=DIRECTION('ref_axis',(0.,0.349194145719507,0.93705039810846));
#30850=DIRECTION('',(1.,0.,0.));
#30851=DIRECTION('center_axis',(1.,0.,0.));
#30852=DIRECTION('ref_axis',(0.,0.349194145719507,0.93705039810846));
#30853=DIRECTION('',(1.,0.,0.));
#30854=DIRECTION('center_axis',(1.,0.,0.));
#30855=DIRECTION('ref_axis',(0.,0.349194145719507,0.93705039810846));
#30856=DIRECTION('',(1.,0.,0.));
#30857=DIRECTION('center_axis',(-1.,0.,0.));
#30858=DIRECTION('ref_axis',(0.,0.,1.));
#30859=DIRECTION('center_axis',(1.,0.,0.));
#30860=DIRECTION('ref_axis',(0.,-0.349194147217983,0.937050397550049));
#30861=DIRECTION('',(1.,0.,0.));
#30862=DIRECTION('center_axis',(1.,0.,0.));
#30863=DIRECTION('ref_axis',(0.,0.,1.));
#30864=DIRECTION('center_axis',(1.,0.,0.));
#30865=DIRECTION('ref_axis',(0.,-0.349194147217983,0.937050397550049));
#30866=DIRECTION('',(1.,0.,0.));
#30867=DIRECTION('center_axis',(1.,0.,0.));
#30868=DIRECTION('ref_axis',(0.,0.,1.));
#30869=DIRECTION('center_axis',(1.,0.,0.));
#30870=DIRECTION('ref_axis',(0.,-0.349194147217983,0.937050397550049));
#30871=DIRECTION('',(1.,0.,0.));
#30872=DIRECTION('center_axis',(1.,0.,0.));
#30873=DIRECTION('ref_axis',(0.,-0.509892608781802,0.86023806443896));
#30874=DIRECTION('',(1.,0.,0.));
#30875=DIRECTION('center_axis',(1.,0.,0.));
#30876=DIRECTION('ref_axis',(0.,0.,1.));
#30877=DIRECTION('center_axis',(0.,0.,-1.));
#30878=DIRECTION('ref_axis',(0.939338961794584,0.342990254751753,0.));
#30879=DIRECTION('',(0.,0.,-1.));
#30880=DIRECTION('center_axis',(0.,0.,1.));
#30881=DIRECTION('ref_axis',(1.,0.,0.));
#30882=DIRECTION('center_axis',(0.,0.,-1.));
#30883=DIRECTION('ref_axis',(0.939338961794584,0.342990254751753,0.));
#30884=DIRECTION('',(0.,0.,-1.));
#30885=DIRECTION('center_axis',(0.,0.,-1.));
#30886=DIRECTION('ref_axis',(0.939338961794584,0.342990254751753,0.));
#30887=DIRECTION('',(0.,0.,-1.));
#30888=DIRECTION('center_axis',(0.,0.,-1.));
#30889=DIRECTION('ref_axis',(0.939338961794584,0.342990254751753,0.));
#30890=DIRECTION('',(0.,0.,-1.));
#30891=DIRECTION('center_axis',(0.,0.,-1.));
#30892=DIRECTION('ref_axis',(0.939338961794584,0.342990254751753,0.));
#30893=DIRECTION('',(0.,0.,-1.));
#30894=DIRECTION('center_axis',(0.,0.,-1.));
#30895=DIRECTION('ref_axis',(0.939338961794584,0.342990254751753,0.));
#30896=DIRECTION('',(0.,0.,-1.));
#30897=DIRECTION('center_axis',(0.,0.,-1.));
#30898=DIRECTION('ref_axis',(0.939338961794584,0.342990254751753,0.));
#30899=DIRECTION('',(0.,0.,-1.));
#30900=DIRECTION('center_axis',(0.,0.,-1.));
#30901=DIRECTION('ref_axis',(0.939338961794584,0.342990254751753,0.));
#30902=DIRECTION('',(0.,0.,-1.));
#30903=DIRECTION('center_axis',(0.,0.,-1.));
#30904=DIRECTION('ref_axis',(0.939338961794584,0.342990254751753,0.));
#30905=DIRECTION('',(0.,0.,-1.));
#30906=DIRECTION('center_axis',(0.,0.,-1.));
#30907=DIRECTION('ref_axis',(0.939338961794584,0.342990254751753,0.));
#30908=DIRECTION('',(0.,0.,-1.));
#30909=DIRECTION('center_axis',(0.,0.,-1.));
#30910=DIRECTION('ref_axis',(0.939338961794584,0.342990254751753,0.));
#30911=DIRECTION('',(0.,0.,-1.));
#30912=DIRECTION('center_axis',(0.,0.,-1.));
#30913=DIRECTION('ref_axis',(0.939338961794584,0.342990254751753,0.));
#30914=DIRECTION('',(0.,0.,-1.));
#30915=DIRECTION('center_axis',(0.,0.,-1.));
#30916=DIRECTION('ref_axis',(0.939338961794584,0.342990254751753,0.));
#30917=DIRECTION('',(0.,0.,-1.));
#30918=DIRECTION('center_axis',(0.,0.,-1.));
#30919=DIRECTION('ref_axis',(0.939338961794584,0.342990254751753,0.));
#30920=DIRECTION('',(0.,0.,-1.));
#30921=DIRECTION('center_axis',(0.,0.,-1.));
#30922=DIRECTION('ref_axis',(0.939338961794584,0.342990254751753,0.));
#30923=DIRECTION('',(0.,0.,-1.));
#30924=DIRECTION('center_axis',(0.,0.,-1.));
#30925=DIRECTION('ref_axis',(0.939338961794584,0.342990254751753,0.));
#30926=DIRECTION('',(0.,0.,-1.));
#30927=DIRECTION('center_axis',(0.,0.,-1.));
#30928=DIRECTION('ref_axis',(0.939338961794584,0.342990254751753,0.));
#30929=DIRECTION('',(0.,0.,-1.));
#30930=DIRECTION('center_axis',(0.,0.,-1.));
#30931=DIRECTION('ref_axis',(0.939338961794584,0.342990254751753,0.));
#30932=DIRECTION('',(0.,0.,-1.));
#30933=DIRECTION('center_axis',(0.,0.,-1.));
#30934=DIRECTION('ref_axis',(0.939338961794584,0.342990254751753,0.));
#30935=DIRECTION('',(0.,0.,-1.));
#30936=DIRECTION('center_axis',(0.,0.,-1.));
#30937=DIRECTION('ref_axis',(0.939338961794584,0.342990254751753,0.));
#30938=DIRECTION('',(0.,0.,-1.));
#30939=DIRECTION('center_axis',(0.,0.,-1.));
#30940=DIRECTION('ref_axis',(0.939338961794584,0.342990254751753,0.));
#30941=DIRECTION('',(0.,0.,-1.));
#30942=DIRECTION('center_axis',(0.,0.,-1.));
#30943=DIRECTION('ref_axis',(0.939338961794584,0.342990254751753,0.));
#30944=DIRECTION('',(0.,0.,-1.));
#30945=DIRECTION('center_axis',(0.,0.,-1.));
#30946=DIRECTION('ref_axis',(0.939338961794584,0.342990254751753,0.));
#30947=DIRECTION('',(0.,0.,-1.));
#30948=DIRECTION('center_axis',(0.,0.,-1.));
#30949=DIRECTION('ref_axis',(0.939338961794584,0.342990254751753,0.));
#30950=DIRECTION('',(0.,0.,-1.));
#30951=DIRECTION('center_axis',(0.,0.,-1.));
#30952=DIRECTION('ref_axis',(0.939338961794584,0.342990254751753,0.));
#30953=DIRECTION('',(0.,0.,-1.));
#30954=DIRECTION('center_axis',(0.,0.,-1.));
#30955=DIRECTION('ref_axis',(0.939338961794584,0.342990254751753,0.));
#30956=DIRECTION('',(0.,0.,-1.));
#30957=DIRECTION('center_axis',(0.,0.,-1.));
#30958=DIRECTION('ref_axis',(0.939338961794584,0.342990254751753,0.));
#30959=DIRECTION('',(0.,0.,-1.));
#30960=DIRECTION('center_axis',(0.,0.,1.));
#30961=DIRECTION('ref_axis',(1.,0.,0.));
#30962=DIRECTION('center_axis',(0.,0.,-1.));
#30963=DIRECTION('ref_axis',(0.93933894663973,0.342990296255976,0.));
#30964=DIRECTION('',(0.,0.,-1.));
#30965=DIRECTION('center_axis',(0.,0.,1.));
#30966=DIRECTION('ref_axis',(1.,0.,0.));
#30967=DIRECTION('center_axis',(0.,0.,-1.));
#30968=DIRECTION('ref_axis',(0.93933894663973,0.342990296255976,0.));
#30969=DIRECTION('',(0.,0.,-1.));
#30970=DIRECTION('center_axis',(0.,0.,-1.));
#30971=DIRECTION('ref_axis',(0.93933894663973,0.342990296255976,0.));
#30972=DIRECTION('',(0.,0.,-1.));
#30973=DIRECTION('center_axis',(0.,0.,-1.));
#30974=DIRECTION('ref_axis',(0.93933894663973,0.342990296255976,0.));
#30975=DIRECTION('',(0.,0.,-1.));
#30976=DIRECTION('center_axis',(0.,0.,-1.));
#30977=DIRECTION('ref_axis',(0.93933894663973,0.342990296255976,0.));
#30978=DIRECTION('',(0.,0.,-1.));
#30979=DIRECTION('center_axis',(0.,0.,-1.));
#30980=DIRECTION('ref_axis',(0.93933894663973,0.342990296255976,0.));
#30981=DIRECTION('',(0.,0.,-1.));
#30982=DIRECTION('center_axis',(0.,0.,-1.));
#30983=DIRECTION('ref_axis',(0.93933894663973,0.342990296255976,0.));
#30984=DIRECTION('',(0.,0.,-1.));
#30985=DIRECTION('center_axis',(0.,0.,-1.));
#30986=DIRECTION('ref_axis',(0.93933894663973,0.342990296255976,0.));
#30987=DIRECTION('',(0.,0.,-1.));
#30988=DIRECTION('center_axis',(0.,0.,-1.));
#30989=DIRECTION('ref_axis',(0.93933894663973,0.342990296255976,0.));
#30990=DIRECTION('',(0.,0.,-1.));
#30991=DIRECTION('center_axis',(0.,0.,-1.));
#30992=DIRECTION('ref_axis',(0.93933894663973,0.342990296255976,0.));
#30993=DIRECTION('',(0.,0.,-1.));
#30994=DIRECTION('center_axis',(0.,0.,-1.));
#30995=DIRECTION('ref_axis',(0.93933894663973,0.342990296255976,0.));
#30996=DIRECTION('',(0.,0.,-1.));
#30997=DIRECTION('center_axis',(0.,0.,-1.));
#30998=DIRECTION('ref_axis',(0.93933894663973,0.342990296255976,0.));
#30999=DIRECTION('',(0.,0.,-1.));
#31000=DIRECTION('center_axis',(0.,0.,-1.));
#31001=DIRECTION('ref_axis',(0.93933894663973,0.342990296255976,0.));
#31002=DIRECTION('',(0.,0.,-1.));
#31003=DIRECTION('center_axis',(0.,0.,-1.));
#31004=DIRECTION('ref_axis',(0.93933894663973,0.342990296255976,0.));
#31005=DIRECTION('',(0.,0.,-1.));
#31006=DIRECTION('center_axis',(0.,0.,-1.));
#31007=DIRECTION('ref_axis',(0.93933894663973,0.342990296255976,0.));
#31008=DIRECTION('',(0.,0.,-1.));
#31009=DIRECTION('center_axis',(0.,0.,-1.));
#31010=DIRECTION('ref_axis',(0.93933894663973,0.342990296255976,0.));
#31011=DIRECTION('',(0.,0.,-1.));
#31012=DIRECTION('center_axis',(0.,0.,-1.));
#31013=DIRECTION('ref_axis',(0.93933894663973,0.342990296255976,0.));
#31014=DIRECTION('',(0.,0.,-1.));
#31015=DIRECTION('center_axis',(0.,0.,-1.));
#31016=DIRECTION('ref_axis',(0.93933894663973,0.342990296255976,0.));
#31017=DIRECTION('',(0.,0.,-1.));
#31018=DIRECTION('center_axis',(0.,0.,-1.));
#31019=DIRECTION('ref_axis',(0.93933894663973,0.342990296255976,0.));
#31020=DIRECTION('',(0.,0.,-1.));
#31021=DIRECTION('center_axis',(0.,0.,-1.));
#31022=DIRECTION('ref_axis',(0.93933894663973,0.342990296255976,0.));
#31023=DIRECTION('',(0.,0.,-1.));
#31024=DIRECTION('center_axis',(0.,0.,-1.));
#31025=DIRECTION('ref_axis',(0.93933894663973,0.342990296255976,0.));
#31026=DIRECTION('',(0.,0.,-1.));
#31027=DIRECTION('center_axis',(0.,0.,-1.));
#31028=DIRECTION('ref_axis',(0.93933894663973,0.342990296255976,0.));
#31029=DIRECTION('',(0.,0.,-1.));
#31030=DIRECTION('center_axis',(0.,0.,-1.));
#31031=DIRECTION('ref_axis',(0.93933894663973,0.342990296255976,0.));
#31032=DIRECTION('',(0.,0.,-1.));
#31033=DIRECTION('center_axis',(0.,0.,-1.));
#31034=DIRECTION('ref_axis',(0.93933894663973,0.342990296255976,0.));
#31035=DIRECTION('',(0.,0.,-1.));
#31036=DIRECTION('center_axis',(0.,0.,-1.));
#31037=DIRECTION('ref_axis',(0.93933894663973,0.342990296255976,0.));
#31038=DIRECTION('',(0.,0.,-1.));
#31039=DIRECTION('center_axis',(0.,0.,-1.));
#31040=DIRECTION('ref_axis',(0.93933894663973,0.342990296255976,0.));
#31041=DIRECTION('',(0.,0.,-1.));
#31042=DIRECTION('center_axis',(0.,0.,-1.));
#31043=DIRECTION('ref_axis',(0.93933894663973,0.342990296255976,0.));
#31044=DIRECTION('',(0.,0.,-1.));
#31045=DIRECTION('center_axis',(0.,0.,1.));
#31046=DIRECTION('ref_axis',(1.,0.,0.));
#31047=DIRECTION('center_axis',(0.,0.,-1.));
#31048=DIRECTION('ref_axis',(0.939338946471827,0.342990296715807,0.));
#31049=DIRECTION('',(0.,0.,-1.));
#31050=DIRECTION('center_axis',(0.,0.,1.));
#31051=DIRECTION('ref_axis',(1.,0.,0.));
#31052=DIRECTION('center_axis',(0.,0.,-1.));
#31053=DIRECTION('ref_axis',(0.939338946471827,0.342990296715807,0.));
#31054=DIRECTION('',(0.,0.,-1.));
#31055=DIRECTION('center_axis',(0.,0.,-1.));
#31056=DIRECTION('ref_axis',(0.939338946471827,0.342990296715807,0.));
#31057=DIRECTION('',(0.,0.,-1.));
#31058=DIRECTION('center_axis',(0.,0.,-1.));
#31059=DIRECTION('ref_axis',(0.939338946471827,0.342990296715807,0.));
#31060=DIRECTION('',(0.,0.,-1.));
#31061=DIRECTION('center_axis',(0.,0.,-1.));
#31062=DIRECTION('ref_axis',(0.939338946471827,0.342990296715807,0.));
#31063=DIRECTION('',(0.,0.,-1.));
#31064=DIRECTION('center_axis',(0.,0.,-1.));
#31065=DIRECTION('ref_axis',(0.939338946471827,0.342990296715807,0.));
#31066=DIRECTION('',(0.,0.,-1.));
#31067=DIRECTION('center_axis',(0.,0.,-1.));
#31068=DIRECTION('ref_axis',(0.939338946471827,0.342990296715807,0.));
#31069=DIRECTION('',(0.,0.,-1.));
#31070=DIRECTION('center_axis',(0.,0.,-1.));
#31071=DIRECTION('ref_axis',(0.939338946471827,0.342990296715807,0.));
#31072=DIRECTION('',(0.,0.,-1.));
#31073=DIRECTION('center_axis',(0.,0.,-1.));
#31074=DIRECTION('ref_axis',(0.939338946471827,0.342990296715807,0.));
#31075=DIRECTION('',(0.,0.,-1.));
#31076=DIRECTION('center_axis',(0.,0.,-1.));
#31077=DIRECTION('ref_axis',(0.939338946471827,0.342990296715807,0.));
#31078=DIRECTION('',(0.,0.,-1.));
#31079=DIRECTION('center_axis',(0.,0.,-1.));
#31080=DIRECTION('ref_axis',(0.939338946471827,0.342990296715807,0.));
#31081=DIRECTION('',(0.,0.,-1.));
#31082=DIRECTION('center_axis',(0.,0.,-1.));
#31083=DIRECTION('ref_axis',(0.939338946471827,0.342990296715807,0.));
#31084=DIRECTION('',(0.,0.,-1.));
#31085=DIRECTION('center_axis',(0.,0.,-1.));
#31086=DIRECTION('ref_axis',(0.939338946471827,0.342990296715807,0.));
#31087=DIRECTION('',(0.,0.,-1.));
#31088=DIRECTION('center_axis',(0.,0.,-1.));
#31089=DIRECTION('ref_axis',(0.939338946471827,0.342990296715807,0.));
#31090=DIRECTION('',(0.,0.,-1.));
#31091=DIRECTION('center_axis',(0.,0.,-1.));
#31092=DIRECTION('ref_axis',(0.939338946471827,0.342990296715807,0.));
#31093=DIRECTION('',(0.,0.,-1.));
#31094=DIRECTION('center_axis',(0.,0.,-1.));
#31095=DIRECTION('ref_axis',(0.939338946471827,0.342990296715807,0.));
#31096=DIRECTION('',(0.,0.,-1.));
#31097=DIRECTION('center_axis',(0.,0.,-1.));
#31098=DIRECTION('ref_axis',(0.939338946471827,0.342990296715807,0.));
#31099=DIRECTION('',(0.,0.,-1.));
#31100=DIRECTION('center_axis',(0.,0.,-1.));
#31101=DIRECTION('ref_axis',(0.939338946471827,0.342990296715807,0.));
#31102=DIRECTION('',(0.,0.,-1.));
#31103=DIRECTION('center_axis',(0.,0.,-1.));
#31104=DIRECTION('ref_axis',(0.939338946471827,0.342990296715807,0.));
#31105=DIRECTION('',(0.,0.,-1.));
#31106=DIRECTION('center_axis',(0.,0.,-1.));
#31107=DIRECTION('ref_axis',(0.939338946471827,0.342990296715807,0.));
#31108=DIRECTION('',(0.,0.,-1.));
#31109=DIRECTION('center_axis',(0.,0.,-1.));
#31110=DIRECTION('ref_axis',(0.939338946471827,0.342990296715807,0.));
#31111=DIRECTION('',(0.,0.,-1.));
#31112=DIRECTION('center_axis',(0.,0.,-1.));
#31113=DIRECTION('ref_axis',(0.939338946471827,0.342990296715807,0.));
#31114=DIRECTION('',(0.,0.,-1.));
#31115=DIRECTION('center_axis',(0.,0.,-1.));
#31116=DIRECTION('ref_axis',(0.939338946471827,0.342990296715807,0.));
#31117=DIRECTION('',(0.,0.,-1.));
#31118=DIRECTION('center_axis',(0.,0.,-1.));
#31119=DIRECTION('ref_axis',(0.939338946471827,0.342990296715807,0.));
#31120=DIRECTION('',(0.,0.,-1.));
#31121=DIRECTION('center_axis',(0.,0.,-1.));
#31122=DIRECTION('ref_axis',(0.939338946471827,0.342990296715807,0.));
#31123=DIRECTION('',(0.,0.,-1.));
#31124=DIRECTION('center_axis',(0.,0.,-1.));
#31125=DIRECTION('ref_axis',(0.939338946471827,0.342990296715807,0.));
#31126=DIRECTION('',(0.,0.,-1.));
#31127=DIRECTION('center_axis',(0.,0.,-1.));
#31128=DIRECTION('ref_axis',(0.939338946471827,0.342990296715807,0.));
#31129=DIRECTION('',(0.,0.,-1.));
#31130=DIRECTION('center_axis',(0.,0.,1.));
#31131=DIRECTION('ref_axis',(1.,0.,0.));
#31132=DIRECTION('center_axis',(0.,0.,-1.));
#31133=DIRECTION('ref_axis',(0.939338976758881,0.3429902137694,0.));
#31134=DIRECTION('',(0.,0.,-1.));
#31135=DIRECTION('center_axis',(0.,0.,1.));
#31136=DIRECTION('ref_axis',(1.,0.,0.));
#31137=DIRECTION('center_axis',(0.,0.,-1.));
#31138=DIRECTION('ref_axis',(0.939338976758881,0.3429902137694,0.));
#31139=DIRECTION('',(0.,0.,-1.));
#31140=DIRECTION('center_axis',(0.,0.,-1.));
#31141=DIRECTION('ref_axis',(0.939338976758881,0.3429902137694,0.));
#31142=DIRECTION('',(0.,0.,-1.));
#31143=DIRECTION('center_axis',(0.,0.,-1.));
#31144=DIRECTION('ref_axis',(0.939338976758881,0.3429902137694,0.));
#31145=DIRECTION('',(0.,0.,-1.));
#31146=DIRECTION('center_axis',(0.,0.,-1.));
#31147=DIRECTION('ref_axis',(0.939338976758881,0.3429902137694,0.));
#31148=DIRECTION('',(0.,0.,-1.));
#31149=DIRECTION('center_axis',(0.,0.,-1.));
#31150=DIRECTION('ref_axis',(0.939338976758881,0.3429902137694,0.));
#31151=DIRECTION('',(0.,0.,-1.));
#31152=DIRECTION('center_axis',(0.,0.,-1.));
#31153=DIRECTION('ref_axis',(0.939338976758881,0.3429902137694,0.));
#31154=DIRECTION('',(0.,0.,-1.));
#31155=DIRECTION('center_axis',(0.,0.,-1.));
#31156=DIRECTION('ref_axis',(0.939338976758881,0.3429902137694,0.));
#31157=DIRECTION('',(0.,0.,-1.));
#31158=DIRECTION('center_axis',(0.,0.,-1.));
#31159=DIRECTION('ref_axis',(0.939338976758881,0.3429902137694,0.));
#31160=DIRECTION('',(0.,0.,-1.));
#31161=DIRECTION('center_axis',(0.,0.,-1.));
#31162=DIRECTION('ref_axis',(0.939338976758881,0.3429902137694,0.));
#31163=DIRECTION('',(0.,0.,-1.));
#31164=DIRECTION('center_axis',(0.,0.,-1.));
#31165=DIRECTION('ref_axis',(0.939338976758881,0.3429902137694,0.));
#31166=DIRECTION('',(0.,0.,-1.));
#31167=DIRECTION('center_axis',(0.,0.,-1.));
#31168=DIRECTION('ref_axis',(0.939338976758881,0.3429902137694,0.));
#31169=DIRECTION('',(0.,0.,-1.));
#31170=DIRECTION('center_axis',(0.,0.,-1.));
#31171=DIRECTION('ref_axis',(0.939338976758881,0.3429902137694,0.));
#31172=DIRECTION('',(0.,0.,-1.));
#31173=DIRECTION('center_axis',(0.,0.,-1.));
#31174=DIRECTION('ref_axis',(0.939338976758881,0.3429902137694,0.));
#31175=DIRECTION('',(0.,0.,-1.));
#31176=DIRECTION('center_axis',(0.,0.,-1.));
#31177=DIRECTION('ref_axis',(0.939338976758881,0.3429902137694,0.));
#31178=DIRECTION('',(0.,0.,-1.));
#31179=DIRECTION('center_axis',(0.,0.,-1.));
#31180=DIRECTION('ref_axis',(0.939338976758881,0.3429902137694,0.));
#31181=DIRECTION('',(0.,0.,-1.));
#31182=DIRECTION('center_axis',(0.,0.,-1.));
#31183=DIRECTION('ref_axis',(0.939338976758881,0.3429902137694,0.));
#31184=DIRECTION('',(0.,0.,-1.));
#31185=DIRECTION('center_axis',(0.,0.,-1.));
#31186=DIRECTION('ref_axis',(0.939338976758881,0.3429902137694,0.));
#31187=DIRECTION('',(0.,0.,-1.));
#31188=DIRECTION('center_axis',(0.,0.,-1.));
#31189=DIRECTION('ref_axis',(0.939338976758881,0.3429902137694,0.));
#31190=DIRECTION('',(0.,0.,-1.));
#31191=DIRECTION('center_axis',(0.,0.,-1.));
#31192=DIRECTION('ref_axis',(0.939338976758881,0.3429902137694,0.));
#31193=DIRECTION('',(0.,0.,-1.));
#31194=DIRECTION('center_axis',(0.,0.,-1.));
#31195=DIRECTION('ref_axis',(0.939338976758881,0.3429902137694,0.));
#31196=DIRECTION('',(0.,0.,-1.));
#31197=DIRECTION('center_axis',(0.,0.,-1.));
#31198=DIRECTION('ref_axis',(0.939338976758881,0.3429902137694,0.));
#31199=DIRECTION('',(0.,0.,-1.));
#31200=DIRECTION('center_axis',(0.,0.,-1.));
#31201=DIRECTION('ref_axis',(0.939338976758881,0.3429902137694,0.));
#31202=DIRECTION('',(0.,0.,-1.));
#31203=DIRECTION('center_axis',(0.,0.,-1.));
#31204=DIRECTION('ref_axis',(0.939338976758881,0.3429902137694,0.));
#31205=DIRECTION('',(0.,0.,-1.));
#31206=DIRECTION('center_axis',(0.,0.,-1.));
#31207=DIRECTION('ref_axis',(0.939338976758881,0.3429902137694,0.));
#31208=DIRECTION('',(0.,0.,-1.));
#31209=DIRECTION('center_axis',(0.,0.,-1.));
#31210=DIRECTION('ref_axis',(0.939338976758881,0.3429902137694,0.));
#31211=DIRECTION('',(0.,0.,-1.));
#31212=DIRECTION('center_axis',(0.,0.,-1.));
#31213=DIRECTION('ref_axis',(0.939338976758881,0.3429902137694,0.));
#31214=DIRECTION('',(0.,0.,-1.));
#31215=DIRECTION('center_axis',(0.,0.,1.));
#31216=DIRECTION('ref_axis',(1.,0.,0.));
#31217=DIRECTION('center_axis',(0.,0.,-1.));
#31218=DIRECTION('ref_axis',(0.939338976758881,0.3429902137694,0.));
#31219=DIRECTION('center_axis',(0.,0.,-1.));
#31220=DIRECTION('ref_axis',(0.939338946471827,0.342990296715807,0.));
#31221=DIRECTION('center_axis',(0.,0.,-1.));
#31222=DIRECTION('ref_axis',(0.93933894663973,0.342990296255976,0.));
#31223=DIRECTION('center_axis',(0.,0.,-1.));
#31224=DIRECTION('ref_axis',(0.939338961794584,0.342990254751753,0.));
#31225=DIRECTION('center_axis',(1.,0.,0.));
#31226=DIRECTION('ref_axis',(0.,-0.349194147217983,0.937050397550049));
#31227=DIRECTION('center_axis',(1.,0.,0.));
#31228=DIRECTION('ref_axis',(0.,0.349194145719507,0.93705039810846));
#31229=DIRECTION('center_axis',(-1.,0.,0.));
#31230=DIRECTION('ref_axis',(0.,0.,1.));
#31231=DIRECTION('center_axis',(0.,0.,-1.));
#31232=DIRECTION('ref_axis',(-0.60919368949553,-0.793021467981053,0.));
#31233=DIRECTION('center_axis',(0.,0.,-1.));
#31234=DIRECTION('ref_axis',(-0.609193706391024,-0.793021455002049,0.));
#31235=DIRECTION('center_axis',(0.,0.,-1.));
#31236=DIRECTION('ref_axis',(-0.609193705300279,-0.793021455839952,0.));
#31237=DIRECTION('center_axis',(0.,0.,-1.));
#31238=DIRECTION('ref_axis',(-0.609193654691519,-0.793021494717256,0.));
#31239=DIRECTION('center_axis',(-1.,0.,0.));
#31240=DIRECTION('ref_axis',(0.,0.793547993033681,-0.608507668605924));
#31241=DIRECTION('center_axis',(1.,0.,0.));
#31242=DIRECTION('ref_axis',(0.,-0.793547993282919,-0.608507668280895));
#31243=DIRECTION('center_axis',(0.,0.,1.));
#31244=DIRECTION('ref_axis',(1.,0.,0.));
#31245=DIRECTION('center_axis',(0.,0.,1.));
#31246=DIRECTION('ref_axis',(1.,0.,0.));
#31247=DIRECTION('',(0.,0.,1.));
#31248=DIRECTION('center_axis',(0.,0.,1.));
#31249=DIRECTION('ref_axis',(1.,0.,0.));
#31250=DIRECTION('center_axis',(0.,0.,-1.));
#31251=DIRECTION('ref_axis',(-1.,0.,0.));
#31252=DIRECTION('center_axis',(0.,0.,1.));
#31253=DIRECTION('ref_axis',(1.,0.,0.));
#31254=DIRECTION('center_axis',(0.,0.,1.));
#31255=DIRECTION('ref_axis',(1.,0.,0.));
#31256=DIRECTION('',(0.,0.,-1.));
#31257=DIRECTION('center_axis',(0.,0.,1.));
#31258=DIRECTION('ref_axis',(1.,0.,0.));
#31259=DIRECTION('',(0.,0.,1.));
#31260=DIRECTION('center_axis',(0.,0.,-1.));
#31261=DIRECTION('ref_axis',(-1.,0.,0.));
#31262=DIRECTION('',(0.,-1.,0.));
#31263=DIRECTION('',(-1.,0.,0.));
#31264=DIRECTION('',(0.,-1.,0.));
#31265=DIRECTION('center_axis',(0.,0.,1.));
#31266=DIRECTION('ref_axis',(-0.374029024133323,0.927416998499529,0.));
#31267=DIRECTION('center_axis',(0.,0.,1.));
#31268=DIRECTION('ref_axis',(1.,0.,0.));
#31269=DIRECTION('center_axis',(0.,0.,1.));
#31270=DIRECTION('ref_axis',(1.,0.,0.));
#31271=DIRECTION('',(0.,0.,1.));
#31272=DIRECTION('center_axis',(0.,0.,1.));
#31273=DIRECTION('ref_axis',(1.,0.,0.));
#31274=DIRECTION('center_axis',(0.,0.,-1.));
#31275=DIRECTION('ref_axis',(-1.,0.,0.));
#31276=DIRECTION('center_axis',(0.,0.,1.));
#31277=DIRECTION('ref_axis',(-0.873226700271574,-0.487314200421882,0.));
#31278=DIRECTION('center_axis',(0.,0.,1.));
#31279=DIRECTION('ref_axis',(1.,0.,0.));
#31280=DIRECTION('',(0.,0.,-1.));
#31281=DIRECTION('center_axis',(0.,0.,1.));
#31282=DIRECTION('ref_axis',(1.,0.,0.));
#31283=DIRECTION('',(0.,0.,1.));
#31284=DIRECTION('center_axis',(0.,0.,-1.));
#31285=DIRECTION('ref_axis',(-1.,0.,0.));
#31286=DIRECTION('',(0.,1.,0.));
#31287=DIRECTION('',(-1.,0.,0.));
#31288=DIRECTION('',(0.,1.,0.));
#31289=DIRECTION('center_axis',(0.,0.,1.));
#31290=DIRECTION('ref_axis',(0.914708142118334,0.404115100859181,0.));
#31291=DIRECTION('center_axis',(0.,0.,1.));
#31292=DIRECTION('ref_axis',(1.,0.,0.));
#31293=DIRECTION('center_axis',(0.,0.,1.));
#31294=DIRECTION('ref_axis',(1.,0.,0.));
#31295=DIRECTION('',(0.,0.,1.));
#31296=DIRECTION('center_axis',(0.,0.,1.));
#31297=DIRECTION('ref_axis',(1.,0.,0.));
#31298=DIRECTION('center_axis',(0.,0.,-1.));
#31299=DIRECTION('ref_axis',(-1.,0.,0.));
#31300=DIRECTION('center_axis',(-1.,0.,0.));
#31301=DIRECTION('ref_axis',(0.,1.,0.));
#31302=DIRECTION('',(0.,0.,-1.));
#31303=DIRECTION('',(0.,1.,0.));
#31304=DIRECTION('',(0.,0.,-1.));
#31305=DIRECTION('center_axis',(1.,0.,0.));
#31306=DIRECTION('ref_axis',(0.,-1.,0.));
#31307=DIRECTION('',(0.,-1.,0.));
#31308=DIRECTION('',(0.,0.,-1.));
#31309=DIRECTION('',(0.,1.,0.));
#31310=DIRECTION('',(0.,0.,-1.));
#31311=DIRECTION('center_axis',(0.,1.,0.));
#31312=DIRECTION('ref_axis',(1.,0.,0.));
#31313=DIRECTION('',(1.,0.,0.));
#31314=DIRECTION('',(0.,0.,-1.));
#31315=DIRECTION('',(-1.,0.,0.));
#31316=DIRECTION('center_axis',(0.,0.,1.));
#31317=DIRECTION('ref_axis',(1.,0.,0.));
#31318=DIRECTION('',(0.,1.,0.));
#31319=DIRECTION('center_axis',(0.,0.,1.));
#31320=DIRECTION('ref_axis',(1.,0.,0.));
#31321=DIRECTION('',(-1.,0.,0.));
#31322=DIRECTION('center_axis',(0.,0.,-1.));
#31323=DIRECTION('ref_axis',(-1.,0.,0.));
#31324=DIRECTION('',(0.,1.,0.));
#31325=DIRECTION('center_axis',(0.,0.,-1.));
#31326=DIRECTION('ref_axis',(0.,1.,0.));
#31327=DIRECTION('',(0.987070639057186,-0.160285849379284,0.));
#31328=DIRECTION('center_axis',(0.,0.,-1.));
#31329=DIRECTION('ref_axis',(1.,4.44089209850062E-16,0.));
#31330=DIRECTION('',(0.,-1.,0.));
#31331=DIRECTION('',(-1.,0.,0.));
#31332=DIRECTION('',(0.,-1.,0.));
#31333=DIRECTION('',(1.,0.,0.));
#31334=DIRECTION('',(0.,-1.,0.));
#31335=DIRECTION('center_axis',(0.,0.,-1.));
#31336=DIRECTION('ref_axis',(0.,-1.,0.));
#31337=DIRECTION('',(-1.,3.69197497485193E-16,0.));
#31338=DIRECTION('center_axis',(0.,0.,-1.));
#31339=DIRECTION('ref_axis',(-1.,0.,0.));
#31340=DIRECTION('',(0.,1.,0.));
#31341=DIRECTION('',(1.,0.,0.));
#31342=DIRECTION('',(0.,1.,0.));
#31343=DIRECTION('',(-1.,0.,0.));
#31344=DIRECTION('',(0.,1.,0.));
#31345=DIRECTION('center_axis',(0.,0.,-1.));
#31346=DIRECTION('ref_axis',(0.,1.,0.));
#31347=DIRECTION('',(0.987070639057186,0.160285849379284,0.));
#31348=DIRECTION('center_axis',(0.,0.,-1.));
#31349=DIRECTION('ref_axis',(1.,0.,0.));
#31350=DIRECTION('',(0.,-1.,0.));
#31351=DIRECTION('center_axis',(0.,0.,-1.));
#31352=DIRECTION('ref_axis',(0.,-1.,0.));
#31353=DIRECTION('',(-1.,0.,0.));
#31354=DIRECTION('center_axis',(0.,0.,1.));
#31355=DIRECTION('ref_axis',(0.,1.,0.));
#31356=DIRECTION('center_axis',(0.,0.,1.));
#31357=DIRECTION('ref_axis',(1.,0.,0.));
#31358=DIRECTION('center_axis',(0.,0.,1.));
#31359=DIRECTION('ref_axis',(1.,0.,0.));
#31360=DIRECTION('center_axis',(0.,0.,1.));
#31361=DIRECTION('ref_axis',(0.,1.,0.));
#31362=DIRECTION('',(0.,-1.,0.));
#31363=DIRECTION('',(-1.,0.,0.));
#31364=DIRECTION('',(0.,1.,0.));
#31365=DIRECTION('',(-1.,0.,0.));
#31366=DIRECTION('center_axis',(0.,-1.,0.));
#31367=DIRECTION('ref_axis',(0.,0.,1.));
#31368=DIRECTION('',(0.,0.,-1.));
#31369=DIRECTION('',(0.,0.,1.));
#31370=DIRECTION('',(-1.,0.,0.));
#31371=DIRECTION('center_axis',(0.,0.,1.));
#31372=DIRECTION('ref_axis',(0.,1.,0.));
#31373=DIRECTION('',(0.,-1.,0.));
#31374=DIRECTION('',(0.,1.,0.));
#31375=DIRECTION('',(-1.,0.,0.));
#31376=DIRECTION('center_axis',(0.,-0.894427190999916,-0.447213595499957));
#31377=DIRECTION('ref_axis',(0.,-0.447213595499957,0.894427190999916));
#31378=DIRECTION('',(0.,0.447213595499957,-0.894427190999916));
#31379=DIRECTION('',(0.,-0.447213595499957,0.894427190999916));
#31380=DIRECTION('',(-1.,0.,0.));
#31381=DIRECTION('center_axis',(0.,0.894427190999916,-0.447213595499957));
#31382=DIRECTION('ref_axis',(0.,-0.447213595499957,-0.894427190999916));
#31383=DIRECTION('',(0.,0.447213595499957,0.894427190999916));
#31384=DIRECTION('',(0.,-0.447213595499957,-0.894427190999916));
#31385=DIRECTION('',(-1.,0.,0.));
#31386=DIRECTION('center_axis',(0.,0.,1.));
#31387=DIRECTION('ref_axis',(0.,1.,0.));
#31388=DIRECTION('',(0.,-1.,0.));
#31389=DIRECTION('',(0.,1.,0.));
#31390=DIRECTION('',(-1.,0.,0.));
#31391=DIRECTION('center_axis',(0.,1.,0.));
#31392=DIRECTION('ref_axis',(0.,0.,-1.));
#31393=DIRECTION('',(0.,0.,1.));
#31394=DIRECTION('',(0.,0.,-1.));
#31395=DIRECTION('center_axis',(1.,0.,0.));
#31396=DIRECTION('ref_axis',(0.,0.,1.));
#31397=DIRECTION('center_axis',(1.,0.,0.));
#31398=DIRECTION('ref_axis',(0.,0.,1.));
#31399=DIRECTION('',(1.,0.,0.));
#31400=DIRECTION('center_axis',(-1.,0.,0.));
#31401=DIRECTION('ref_axis',(0.,0.,1.));
#31402=DIRECTION('center_axis',(-1.,0.,0.));
#31403=DIRECTION('ref_axis',(0.,0.,1.));
#31404=DIRECTION('center_axis',(1.,0.,0.));
#31405=DIRECTION('ref_axis',(0.,-0.912870929175277,0.408248290463863));
#31406=DIRECTION('center_axis',(-1.,0.,0.));
#31407=DIRECTION('ref_axis',(0.,0.,1.));
#31408=DIRECTION('',(-1.,0.,0.));
#31409=DIRECTION('center_axis',(1.,0.,0.));
#31410=DIRECTION('ref_axis',(0.,0.,1.));
#31411=DIRECTION('',(-1.,0.,0.));
#31412=DIRECTION('center_axis',(0.,0.,-1.));
#31413=DIRECTION('ref_axis',(0.,-1.,0.));
#31414=DIRECTION('',(0.,1.,0.));
#31415=DIRECTION('',(0.,-1.,0.));
#31416=DIRECTION('',(-1.,0.,0.));
#31417=DIRECTION('center_axis',(1.,0.,0.));
#31418=DIRECTION('ref_axis',(0.,0.912870929175277,0.408248290463863));
#31419=DIRECTION('center_axis',(-1.,0.,0.));
#31420=DIRECTION('ref_axis',(0.,0.,1.));
#31421=DIRECTION('center_axis',(1.,0.,0.));
#31422=DIRECTION('ref_axis',(0.,0.,1.));
#31423=DIRECTION('',(-1.,0.,0.));
#31424=DIRECTION('center_axis',(0.,-1.,0.));
#31425=DIRECTION('ref_axis',(0.,0.,1.));
#31426=DIRECTION('',(0.,0.,-1.));
#31427=DIRECTION('',(0.,0.,1.));
#31428=DIRECTION('center_axis',(0.,1.,0.));
#31429=DIRECTION('ref_axis',(0.,0.,-1.));
#31430=DIRECTION('',(0.,0.,1.));
#31431=DIRECTION('',(0.,0.,-1.));
#31432=DIRECTION('center_axis',(-1.,0.,0.));
#31433=DIRECTION('ref_axis',(0.,0.,1.));
#31434=DIRECTION('center_axis',(1.,0.,0.));
#31435=DIRECTION('ref_axis',(0.,0.,1.));
#31436=DIRECTION('center_axis',(1.,0.,0.));
#31437=DIRECTION('ref_axis',(0.,0.,1.));
#31438=DIRECTION('center_axis',(0.,1.,0.));
#31439=DIRECTION('ref_axis',(0.,0.,-1.));
#31440=DIRECTION('',(0.,0.,1.));
#31441=DIRECTION('',(-1.,0.,0.));
#31442=DIRECTION('',(0.,0.,-1.));
#31443=DIRECTION('',(-1.,0.,0.));
#31444=DIRECTION('center_axis',(0.,0.,-1.));
#31445=DIRECTION('ref_axis',(0.,-1.,0.));
#31446=DIRECTION('',(0.,1.,0.));
#31447=DIRECTION('',(0.,-1.,0.));
#31448=DIRECTION('',(-1.,0.,0.));
#31449=DIRECTION('center_axis',(0.,0.894427190999916,0.447213595499958));
#31450=DIRECTION('ref_axis',(0.,0.447213595499958,-0.894427190999916));
#31451=DIRECTION('',(0.,-0.447213595499958,0.894427190999916));
#31452=DIRECTION('',(0.,0.447213595499958,-0.894427190999916));
#31453=DIRECTION('',(-1.,0.,0.));
#31454=DIRECTION('center_axis',(0.,-0.894427190999916,0.447213595499958));
#31455=DIRECTION('ref_axis',(0.,0.447213595499958,0.894427190999916));
#31456=DIRECTION('',(0.,-0.447213595499958,-0.894427190999916));
#31457=DIRECTION('',(0.,0.447213595499958,0.894427190999916));
#31458=DIRECTION('',(-1.,0.,0.));
#31459=DIRECTION('center_axis',(0.,0.,-1.));
#31460=DIRECTION('ref_axis',(0.,-1.,0.));
#31461=DIRECTION('',(0.,1.,0.));
#31462=DIRECTION('',(0.,-1.,0.));
#31463=DIRECTION('',(-1.,0.,0.));
#31464=DIRECTION('center_axis',(0.,-1.,0.));
#31465=DIRECTION('ref_axis',(0.,0.,1.));
#31466=DIRECTION('',(0.,0.,-1.));
#31467=DIRECTION('',(0.,0.,1.));
#31468=DIRECTION('',(-1.,0.,0.));
#31469=DIRECTION('center_axis',(0.,0.,-1.));
#31470=DIRECTION('ref_axis',(0.,-1.,0.));
#31471=DIRECTION('',(0.,1.,0.));
#31472=DIRECTION('',(0.,-1.,0.));
#31473=DIRECTION('center_axis',(1.,0.,0.));
#31474=DIRECTION('ref_axis',(0.,0.,1.));
#31475=DIRECTION('center_axis',(1.,0.,0.));
#31476=DIRECTION('ref_axis',(0.,0.,1.));
#31477=DIRECTION('',(1.,0.,0.));
#31478=DIRECTION('center_axis',(-1.,0.,0.));
#31479=DIRECTION('ref_axis',(0.,0.,1.));
#31480=DIRECTION('center_axis',(-1.,0.,0.));
#31481=DIRECTION('ref_axis',(0.,0.,1.));
#31482=DIRECTION('center_axis',(1.,0.,0.));
#31483=DIRECTION('ref_axis',(0.,-1.,0.));
#31484=DIRECTION('center_axis',(1.,0.,0.));
#31485=DIRECTION('ref_axis',(0.,-1.,0.));
#31486=DIRECTION('center_axis',(1.,0.,0.));
#31487=DIRECTION('ref_axis',(0.,0.,1.));
#31488=DIRECTION('center_axis',(1.,0.,0.));
#31489=DIRECTION('ref_axis',(0.,0.,1.));
#31490=DIRECTION('',(1.,0.,0.));
#31491=DIRECTION('center_axis',(-1.,0.,0.));
#31492=DIRECTION('ref_axis',(0.,0.,1.));
#31493=DIRECTION('center_axis',(-1.,0.,0.));
#31494=DIRECTION('ref_axis',(0.,0.,1.));
#31495=DIRECTION('center_axis',(1.,0.,0.));
#31496=DIRECTION('ref_axis',(0.,0.,1.));
#31497=DIRECTION('center_axis',(1.,0.,0.));
#31498=DIRECTION('ref_axis',(0.,0.,1.));
#31499=DIRECTION('',(1.,0.,0.));
#31500=DIRECTION('center_axis',(-1.,0.,0.));
#31501=DIRECTION('ref_axis',(0.,0.,1.));
#31502=DIRECTION('center_axis',(1.,0.,0.));
#31503=DIRECTION('ref_axis',(0.,-0.912870929175277,0.408248290463863));
#31504=DIRECTION('center_axis',(1.,0.,0.));
#31505=DIRECTION('ref_axis',(0.,0.,1.));
#31506=DIRECTION('',(1.,0.,0.));
#31507=DIRECTION('center_axis',(1.,0.,0.));
#31508=DIRECTION('ref_axis',(0.,0.,1.));
#31509=DIRECTION('',(1.,0.,0.));
#31510=DIRECTION('center_axis',(0.,0.,1.));
#31511=DIRECTION('ref_axis',(0.,-1.,0.));
#31512=DIRECTION('',(0.,-1.,0.));
#31513=DIRECTION('',(1.,0.,0.));
#31514=DIRECTION('',(0.,-1.,0.));
#31515=DIRECTION('center_axis',(1.,0.,0.));
#31516=DIRECTION('ref_axis',(0.,0.912870929175277,0.408248290463863));
#31517=DIRECTION('center_axis',(1.,0.,0.));
#31518=DIRECTION('ref_axis',(0.,0.,1.));
#31519=DIRECTION('',(1.,0.,0.));
#31520=DIRECTION('center_axis',(1.,0.,0.));
#31521=DIRECTION('ref_axis',(0.,0.,1.));
#31522=DIRECTION('center_axis',(0.,1.,0.));
#31523=DIRECTION('ref_axis',(0.,0.,1.));
#31524=DIRECTION('',(0.,0.,1.));
#31525=DIRECTION('',(0.,0.,1.));
#31526=DIRECTION('center_axis',(0.,-1.,0.));
#31527=DIRECTION('ref_axis',(0.,0.,-1.));
#31528=DIRECTION('',(0.,0.,-1.));
#31529=DIRECTION('',(0.,0.,-1.));
#31530=DIRECTION('center_axis',(-1.,0.,0.));
#31531=DIRECTION('ref_axis',(0.,0.,1.));
#31532=DIRECTION('center_axis',(-1.,0.,0.));
#31533=DIRECTION('ref_axis',(0.,0.,1.));
#31534=DIRECTION('center_axis',(-1.,0.,0.));
#31535=DIRECTION('ref_axis',(0.,0.,1.));
#31536=DIRECTION('center_axis',(0.,-1.,0.));
#31537=DIRECTION('ref_axis',(0.,0.,-1.));
#31538=DIRECTION('',(0.,0.,-1.));
#31539=DIRECTION('',(1.,0.,0.));
#31540=DIRECTION('',(0.,0.,-1.));
#31541=DIRECTION('',(1.,0.,0.));
#31542=DIRECTION('center_axis',(0.,0.,1.));
#31543=DIRECTION('ref_axis',(0.,-1.,0.));
#31544=DIRECTION('',(0.,-1.,0.));
#31545=DIRECTION('',(1.,0.,0.));
#31546=DIRECTION('',(0.,-1.,0.));
#31547=DIRECTION('center_axis',(0.,-0.894427190999916,-0.447213595499958));
#31548=DIRECTION('ref_axis',(0.,0.447213595499958,-0.894427190999916));
#31549=DIRECTION('',(0.,0.447213595499958,-0.894427190999916));
#31550=DIRECTION('',(1.,0.,0.));
#31551=DIRECTION('',(0.,0.447213595499958,-0.894427190999916));
#31552=DIRECTION('center_axis',(0.,0.894427190999916,-0.447213595499958));
#31553=DIRECTION('ref_axis',(0.,0.447213595499958,0.894427190999916));
#31554=DIRECTION('',(0.,0.447213595499958,0.894427190999916));
#31555=DIRECTION('',(1.,0.,0.));
#31556=DIRECTION('',(0.,0.447213595499958,0.894427190999916));
#31557=DIRECTION('center_axis',(0.,0.,1.));
#31558=DIRECTION('ref_axis',(0.,-1.,0.));
#31559=DIRECTION('',(0.,-1.,0.));
#31560=DIRECTION('',(1.,0.,0.));
#31561=DIRECTION('',(0.,-1.,0.));
#31562=DIRECTION('center_axis',(0.,1.,0.));
#31563=DIRECTION('ref_axis',(0.,0.,1.));
#31564=DIRECTION('',(0.,0.,1.));
#31565=DIRECTION('',(1.,0.,0.));
#31566=DIRECTION('',(0.,0.,1.));
#31567=DIRECTION('center_axis',(0.,0.,1.));
#31568=DIRECTION('ref_axis',(0.,-1.,0.));
#31569=DIRECTION('',(0.,-1.,0.));
#31570=DIRECTION('',(0.,-1.,0.));
#31571=DIRECTION('center_axis',(1.,0.,0.));
#31572=DIRECTION('ref_axis',(0.,0.,1.));
#31573=DIRECTION('center_axis',(1.,0.,0.));
#31574=DIRECTION('ref_axis',(0.,0.,1.));
#31575=DIRECTION('',(1.,0.,0.));
#31576=DIRECTION('center_axis',(1.,0.,0.));
#31577=DIRECTION('ref_axis',(0.,0.,1.));
#31578=DIRECTION('center_axis',(-1.,0.,0.));
#31579=DIRECTION('ref_axis',(0.,0.,1.));
#31580=DIRECTION('center_axis',(0.,0.,-1.));
#31581=DIRECTION('ref_axis',(0.,1.,0.));
#31582=DIRECTION('',(0.,1.,0.));
#31583=DIRECTION('',(1.,0.,0.));
#31584=DIRECTION('',(0.,1.,0.));
#31585=DIRECTION('',(1.,0.,0.));
#31586=DIRECTION('center_axis',(0.,1.,0.));
#31587=DIRECTION('ref_axis',(0.,0.,1.));
#31588=DIRECTION('',(0.,0.,1.));
#31589=DIRECTION('',(1.,0.,0.));
#31590=DIRECTION('',(0.,0.,1.));
#31591=DIRECTION('center_axis',(0.,0.,-1.));
#31592=DIRECTION('ref_axis',(0.,1.,0.));
#31593=DIRECTION('',(0.,1.,0.));
#31594=DIRECTION('',(1.,0.,0.));
#31595=DIRECTION('',(0.,1.,0.));
#31596=DIRECTION('center_axis',(0.,0.894427190999916,0.447213595499957));
#31597=DIRECTION('ref_axis',(0.,-0.447213595499957,0.894427190999916));
#31598=DIRECTION('',(0.,-0.447213595499957,0.894427190999916));
#31599=DIRECTION('',(1.,0.,0.));
#31600=DIRECTION('',(0.,-0.447213595499957,0.894427190999916));
#31601=DIRECTION('center_axis',(0.,-0.894427190999916,0.447213595499957));
#31602=DIRECTION('ref_axis',(0.,-0.447213595499957,-0.894427190999916));
#31603=DIRECTION('',(0.,-0.447213595499957,-0.894427190999916));
#31604=DIRECTION('',(1.,0.,0.));
#31605=DIRECTION('',(0.,-0.447213595499957,-0.894427190999916));
#31606=DIRECTION('center_axis',(0.,0.,-1.));
#31607=DIRECTION('ref_axis',(0.,1.,0.));
#31608=DIRECTION('',(0.,1.,0.));
#31609=DIRECTION('',(1.,0.,0.));
#31610=DIRECTION('',(0.,1.,0.));
#31611=DIRECTION('center_axis',(0.,-1.,0.));
#31612=DIRECTION('ref_axis',(0.,0.,-1.));
#31613=DIRECTION('',(0.,0.,-1.));
#31614=DIRECTION('',(0.,0.,-1.));
#31615=DIRECTION('center_axis',(1.,0.,0.));
#31616=DIRECTION('ref_axis',(0.,0.,1.));
#31617=DIRECTION('center_axis',(1.,0.,0.));
#31618=DIRECTION('ref_axis',(0.,0.,1.));
#31619=DIRECTION('',(1.,0.,0.));
#31620=DIRECTION('center_axis',(1.,0.,0.));
#31621=DIRECTION('ref_axis',(0.,0.,1.));
#31622=DIRECTION('center_axis',(-1.,0.,0.));
#31623=DIRECTION('ref_axis',(0.,0.,1.));
#31624=DIRECTION('center_axis',(-1.,0.,0.));
#31625=DIRECTION('ref_axis',(0.,1.,0.));
#31626=DIRECTION('center_axis',(-1.,0.,0.));
#31627=DIRECTION('ref_axis',(0.,1.,0.));
#31628=DIRECTION('center_axis',(-1.,0.,0.));
#31629=DIRECTION('ref_axis',(0.,1.,0.));
#31630=DIRECTION('',(0.,0.,-1.));
#31631=DIRECTION('',(0.,-1.,0.));
#31632=DIRECTION('',(0.,0.,-1.));
#31633=DIRECTION('center_axis',(-1.,0.,0.));
#31634=DIRECTION('ref_axis',(0.,0.,1.));
#31635=DIRECTION('center_axis',(1.,0.,0.));
#31636=DIRECTION('ref_axis',(0.,0.,1.));
#31637=DIRECTION('',(1.,0.,0.));
#31638=DIRECTION('center_axis',(1.,0.,0.));
#31639=DIRECTION('ref_axis',(0.,0.,1.));
#31640=DIRECTION('center_axis',(-1.,0.,0.));
#31641=DIRECTION('ref_axis',(0.,0.,1.));
#31642=DIRECTION('center_axis',(1.,0.,0.));
#31643=DIRECTION('ref_axis',(0.,0.,1.));
#31644=DIRECTION('',(1.,0.,0.));
#31645=DIRECTION('center_axis',(1.,0.,0.));
#31646=DIRECTION('ref_axis',(0.,0.,1.));
#31647=DIRECTION('center_axis',(-1.,0.,0.));
#31648=DIRECTION('ref_axis',(0.,0.,1.));
#31649=DIRECTION('center_axis',(0.,0.,1.));
#31650=DIRECTION('ref_axis',(1.,0.,0.));
#31651=DIRECTION('',(0.,0.,1.));
#31652=DIRECTION('center_axis',(0.,0.,1.));
#31653=DIRECTION('ref_axis',(1.,0.,0.));
#31654=DIRECTION('center_axis',(0.,0.,-1.));
#31655=DIRECTION('ref_axis',(-1.,0.,0.));
#31656=DIRECTION('center_axis',(0.,0.,1.));
#31657=DIRECTION('ref_axis',(1.,0.,0.));
#31658=DIRECTION('',(0.,0.,1.));
#31659=DIRECTION('center_axis',(0.,0.,1.));
#31660=DIRECTION('ref_axis',(1.,0.,0.));
#31661=DIRECTION('center_axis',(0.,0.,-1.));
#31662=DIRECTION('ref_axis',(-1.,0.,0.));
#31663=DIRECTION('center_axis',(1.,0.,0.));
#31664=DIRECTION('ref_axis',(0.,-1.,0.));
#31665=DIRECTION('',(0.,0.,-1.));
#31666=DIRECTION('',(0.,1.,0.));
#31667=DIRECTION('center_axis',(0.,0.,-1.));
#31668=DIRECTION('ref_axis',(0.914708142118334,0.404115100859181,0.));
#31669=DIRECTION('center_axis',(0.,0.,1.));
#31670=DIRECTION('ref_axis',(0.914708142118334,0.404115100859181,0.));
#31671=DIRECTION('center_axis',(0.,0.,-1.));
#31672=DIRECTION('ref_axis',(0.,1.,0.));
#31673=DIRECTION('center_axis',(0.,0.,1.));
#31674=DIRECTION('ref_axis',(0.,1.,0.));
#31675=DIRECTION('',(0.,0.,-1.));
#31676=DIRECTION('center_axis',(0.,-1.,0.));
#31677=DIRECTION('ref_axis',(-1.,0.,0.));
#31678=DIRECTION('',(1.,0.,0.));
#31679=DIRECTION('',(0.,0.,-1.));
#31680=DIRECTION('center_axis',(0.,0.,-1.));
#31681=DIRECTION('ref_axis',(0.,-1.,0.));
#31682=DIRECTION('center_axis',(0.,0.,1.));
#31683=DIRECTION('ref_axis',(0.,-1.,0.));
#31684=DIRECTION('',(0.,0.,-1.));
#31685=DIRECTION('center_axis',(1.,0.,0.));
#31686=DIRECTION('ref_axis',(0.,-1.,0.));
#31687=DIRECTION('',(0.,1.,0.));
#31688=DIRECTION('',(0.,0.,-1.));
#31689=DIRECTION('center_axis',(0.,0.,-1.));
#31690=DIRECTION('ref_axis',(1.,0.,0.));
#31691=DIRECTION('center_axis',(0.,0.,1.));
#31692=DIRECTION('ref_axis',(1.,0.,0.));
#31693=DIRECTION('',(0.,0.,-1.));
#31694=DIRECTION('center_axis',(-0.160285849379284,0.987070639057186,0.));
#31695=DIRECTION('ref_axis',(0.987070639057186,0.160285849379284,0.));
#31696=DIRECTION('',(-0.987070639057186,-0.160285849379284,0.));
#31697=DIRECTION('',(0.,0.,-1.));
#31698=DIRECTION('center_axis',(0.,0.,-1.));
#31699=DIRECTION('ref_axis',(0.,1.,0.));
#31700=DIRECTION('center_axis',(0.,0.,1.));
#31701=DIRECTION('ref_axis',(0.,1.,0.));
#31702=DIRECTION('center_axis',(0.,0.,-1.));
#31703=DIRECTION('ref_axis',(-1.,0.,0.));
#31704=DIRECTION('center_axis',(0.,0.,1.));
#31705=DIRECTION('ref_axis',(-1.,0.,0.));
#31706=DIRECTION('',(0.,0.,-1.));
#31707=DIRECTION('center_axis',(-3.69197497485193E-16,-1.,0.));
#31708=DIRECTION('ref_axis',(-1.,3.69197497485193E-16,0.));
#31709=DIRECTION('',(1.,-3.69197497485193E-16,0.));
#31710=DIRECTION('',(0.,0.,-1.));
#31711=DIRECTION('center_axis',(0.,0.,-1.));
#31712=DIRECTION('ref_axis',(0.,-1.,0.));
#31713=DIRECTION('center_axis',(0.,0.,1.));
#31714=DIRECTION('ref_axis',(0.,-1.,0.));
#31715=DIRECTION('',(0.,0.,-1.));
#31716=DIRECTION('center_axis',(1.,0.,0.));
#31717=DIRECTION('ref_axis',(0.,-1.,0.));
#31718=DIRECTION('',(0.,0.,-1.));
#31719=DIRECTION('',(0.,-1.,0.));
#31720=DIRECTION('center_axis',(0.,0.,-1.));
#31721=DIRECTION('ref_axis',(1.,4.44089209850062E-16,0.));
#31722=DIRECTION('center_axis',(0.,0.,1.));
#31723=DIRECTION('ref_axis',(1.,4.44089209850062E-16,0.));
#31724=DIRECTION('',(0.,0.,-1.));
#31725=DIRECTION('center_axis',(0.160285849379284,0.987070639057186,0.));
#31726=DIRECTION('ref_axis',(0.987070639057186,-0.160285849379284,0.));
#31727=DIRECTION('',(0.987070639057186,-0.160285849379284,0.));
#31728=DIRECTION('',(0.,0.,-1.));
#31729=DIRECTION('center_axis',(0.,0.,-1.));
#31730=DIRECTION('ref_axis',(0.,1.,0.));
#31731=DIRECTION('center_axis',(0.,0.,1.));
#31732=DIRECTION('ref_axis',(0.,1.,0.));
#31733=DIRECTION('',(0.,0.,-1.));
#31734=DIRECTION('center_axis',(-1.,0.,0.));
#31735=DIRECTION('ref_axis',(0.,1.,0.));
#31736=DIRECTION('',(0.,1.,0.));
#31737=DIRECTION('',(0.,0.,-1.));
#31738=DIRECTION('center_axis',(0.,0.,-1.));
#31739=DIRECTION('ref_axis',(-1.,0.,0.));
#31740=DIRECTION('center_axis',(0.,0.,1.));
#31741=DIRECTION('ref_axis',(-1.,0.,0.));
#31742=DIRECTION('',(0.,0.,-1.));
#31743=DIRECTION('center_axis',(0.,-1.,0.));
#31744=DIRECTION('ref_axis',(-1.,0.,0.));
#31745=DIRECTION('',(-1.,0.,0.));
#31746=DIRECTION('',(0.,0.,-1.));
#31747=DIRECTION('center_axis',(0.,0.,-1.));
#31748=DIRECTION('ref_axis',(1.,0.,0.));
#31749=DIRECTION('center_axis',(0.,0.,1.));
#31750=DIRECTION('ref_axis',(1.,0.,0.));
#31751=DIRECTION('',(0.,0.,-1.));
#31752=DIRECTION('center_axis',(-1.,0.,0.));
#31753=DIRECTION('ref_axis',(0.,1.,0.));
#31754=DIRECTION('',(0.,0.,-1.));
#31755=DIRECTION('',(0.,1.,0.));
#31756=DIRECTION('center_axis',(0.,0.,-1.));
#31757=DIRECTION('ref_axis',(-0.374029024133323,0.927416998499529,0.));
#31758=DIRECTION('center_axis',(0.,0.,1.));
#31759=DIRECTION('ref_axis',(-0.374029024133323,0.927416998499529,0.));
#31760=DIRECTION('center_axis',(0.,0.,1.));
#31761=DIRECTION('ref_axis',(1.,0.,0.));
#36294=CARTESIAN_POINT('',(0.,0.,0.));
#36295=CARTESIAN_POINT('Origin',(-26.8463464956315,10.1295,-7.));
#36296=CARTESIAN_POINT('',(-18.1904820161982,14.1758012177496,-3.89721939943572));
#36297=CARTESIAN_POINT('',(-18.0651682165609,14.1759493590362,-3.89710566674782));
#36298=CARTESIAN_POINT('',(-26.8463464956315,14.1758012177496,-3.89721939943572));
#36299=CARTESIAN_POINT('',(-17.734,7.81752421401937,-2.45527019889639));
#36300=CARTESIAN_POINT('Ctrl Pts',(-18.0651682165609,14.1759493590362,-3.89710566674782));
#36301=CARTESIAN_POINT('Ctrl Pts',(-18.0323425743127,13.7488769914328,-3.34120500142468));
#36302=CARTESIAN_POINT('Ctrl Pts',(-17.9607350504285,12.5654944078269,-2.3209180299781));
#36303=CARTESIAN_POINT('Ctrl Pts',(-17.8503456449082,10.2181819306684,-1.69542365644608));
#36304=CARTESIAN_POINT('Ctrl Pts',(-17.772781881636,8.55581177954194,-2.07969166083582));
#36305=CARTESIAN_POINT('Ctrl Pts',(-17.734,7.81752421401937,-2.45527019889639));
#36306=CARTESIAN_POINT('',(-17.734,5.85128156875001,-4.22571665929507));
#36307=CARTESIAN_POINT('Origin',(-17.734,10.1295,-7.));
#36308=CARTESIAN_POINT('Ctrl Pts',(-18.1904820161982,14.1758012177496,-3.89721939943572));
#36309=CARTESIAN_POINT('Ctrl Pts',(-18.1876881222065,14.1394962858778,-3.84987454688103));
#36310=CARTESIAN_POINT('Ctrl Pts',(-18.1848942282147,14.1023624762433,-3.80316978768467));
#36311=CARTESIAN_POINT('Ctrl Pts',(-18.182100334223,14.0644233505464,-3.75713410309268));
#36312=CARTESIAN_POINT('Ctrl Pts',(-18.1751666150798,13.9702682956653,-3.64288549220289));
#36313=CARTESIAN_POINT('Ctrl Pts',(-18.1682328959365,13.8711179308502,-3.53272057308594));
#36314=CARTESIAN_POINT('Ctrl Pts',(-18.1612991767932,13.7673500985625,-3.42706735854301));
#36315=CARTESIAN_POINT('Ctrl Pts',(-18.154366774106,13.6636019679364,-3.32143420362577));
#36316=CARTESIAN_POINT('Ctrl Pts',(-18.1474343714188,13.5552383504529,-3.22031127992504));
#36317=CARTESIAN_POINT('Ctrl Pts',(-18.1405019687316,13.4426745623103,-3.12409038809468));
#36318=CARTESIAN_POINT('Ctrl Pts',(-18.1335693228231,13.3301068249018,-3.02786612038393));
#36319=CARTESIAN_POINT('Ctrl Pts',(-18.1266366769147,13.2133388710388,-2.93654444601234));
#36320=CARTESIAN_POINT('Ctrl Pts',(-18.1197040310062,13.0928201831576,-2.85047779954234));
#36321=CARTESIAN_POINT('Ctrl Pts',(-18.1127717611685,12.9723080329749,-2.76441582187356));
#36322=CARTESIAN_POINT('Ctrl Pts',(-18.1058394913308,12.8480458254471,-2.68360849304181));
#36323=CARTESIAN_POINT('Ctrl Pts',(-18.0989072214931,12.7205131946587,-2.60836572275146));
#36324=CARTESIAN_POINT('Ctrl Pts',(-18.0919734128154,12.5929522539071,-2.53310624991173));
#36325=CARTESIAN_POINT('Ctrl Pts',(-18.0850396041378,12.462119724094,-2.46341397180043));
#36326=CARTESIAN_POINT('Ctrl Pts',(-18.0781057954601,12.3285216260018,-2.39955383811784));
#36327=CARTESIAN_POINT('Ctrl Pts',(-18.0739887600783,12.2491960890059,-2.36163608727149));
#36328=CARTESIAN_POINT('Ctrl Pts',(-18.0698717246966,12.168896016092,-2.32577360896847));
#36329=CARTESIAN_POINT('Ctrl Pts',(-18.0657546893148,12.0877310379076,-2.29201399724091));
#36330=CARTESIAN_POINT('Ctrl Pts',(-18.0588213575568,11.9510444008739,-2.23516080886065));
#36331=CARTESIAN_POINT('Ctrl Pts',(-18.0518880257988,11.8118565702988,-2.18425443407282));
#36332=CARTESIAN_POINT('Ctrl Pts',(-18.0449546940409,11.6707017706744,-2.13949610615628));
#36333=CARTESIAN_POINT('Ctrl Pts',(-18.0380226791153,11.52957378027,-2.09474627909029));
#36334=CARTESIAN_POINT('Ctrl Pts',(-18.0310906641897,11.3864798811559,-2.05614226907002));
#36335=CARTESIAN_POINT('Ctrl Pts',(-18.0241586492642,11.2419704520384,-2.02383576503533));
#36336=CARTESIAN_POINT('Ctrl Pts',(-18.0172263879248,11.0974558860127,-1.99152811259429));
#36337=CARTESIAN_POINT('Ctrl Pts',(-18.0102941265854,10.9515260112177,-1.96551848947931));
#36338=CARTESIAN_POINT('Ctrl Pts',(-18.0033618652459,10.8047429609757,-1.94590780222078));
#36339=CARTESIAN_POINT('Ctrl Pts',(-17.9964299772503,10.6579678158787,-1.92629817111502));
#36340=CARTESIAN_POINT('Ctrl Pts',(-17.9894980892546,10.5103399151234,-1.9130868291269));
#36341=CARTESIAN_POINT('Ctrl Pts',(-17.9825662012589,10.3624281190368,-1.9063229891009));
#36342=CARTESIAN_POINT('Ctrl Pts',(-17.9756327668903,10.2144833266306,-1.89955764019033));
#36343=CARTESIAN_POINT('Ctrl Pts',(-17.9686993325218,10.0662548427467,-1.89924268229057));
#36344=CARTESIAN_POINT('Ctrl Pts',(-17.9617658981532,9.91831378778123,-1.90537524602953));
#36345=CARTESIAN_POINT('Ctrl Pts',(-17.9576469469043,9.8304263195057,-1.90901842338271));
#36346=CARTESIAN_POINT('Ctrl Pts',(-17.9535279956555,9.74264030258537,-1.91493606689122));
#36347=CARTESIAN_POINT('Ctrl Pts',(-17.9494090444066,9.65507506418636,-1.92311887274498));
#36348=CARTESIAN_POINT('Ctrl Pts',(-17.9424753846608,9.50767162774376,-1.93689344499123));
#36349=CARTESIAN_POINT('Ctrl Pts',(-17.9355417249149,9.36084306546452,-1.95709434074805));
#36350=CARTESIAN_POINT('Ctrl Pts',(-17.9286080651691,9.21515569028204,-1.98364918658131));
#36351=CARTESIAN_POINT('Ctrl Pts',(-17.921675723217,9.06949600407137,-2.01019898546813));
#36352=CARTESIAN_POINT('Ctrl Pts',(-17.9147433812648,8.9249773972537,-2.04310026581364));
#36353=CARTESIAN_POINT('Ctrl Pts',(-17.9078110393127,8.78215725526951,-2.08222931317227));
#36354=CARTESIAN_POINT('Ctrl Pts',(-17.9008784555401,8.63933213129698,-2.12135972546763));
#36355=CARTESIAN_POINT('Ctrl Pts',(-17.8939458717674,8.49820591040426,-2.16671825537547));
#36356=CARTESIAN_POINT('Ctrl Pts',(-17.8870132879947,8.35932258344625,-2.21813081380062));
#36357=CARTESIAN_POINT('Ctrl Pts',(-17.8800810809331,8.22044680329677,-2.26954057850861));
#36358=CARTESIAN_POINT('Ctrl Pts',(-17.8731488738714,8.08381398289625,-2.32700359783838));
#36359=CARTESIAN_POINT('Ctrl Pts',(-17.8662166668098,7.94994985065518,-2.39029695679961));
#36360=CARTESIAN_POINT('Ctrl Pts',(-17.8592829213363,7.81605601096829,-2.45360436197322));
#36361=CARTESIAN_POINT('Ctrl Pts',(-17.8523491758629,7.68493238611156,-2.52274455078309));
#36362=CARTESIAN_POINT('Ctrl Pts',(-17.8454154303894,7.55708231303193,-2.59744753083239));
#36363=CARTESIAN_POINT('Ctrl Pts',(-17.8412980867591,7.48116336186096,-2.64180708228259));
#36364=CARTESIAN_POINT('Ctrl Pts',(-17.8371807431287,7.40639825299786,-2.68812726300884));
#36365=CARTESIAN_POINT('Ctrl Pts',(-17.8330633994984,7.33288794460905,-2.73634405566748));
#36366=CARTESIAN_POINT('Ctrl Pts',(-17.8261558247304,7.20956135421445,-2.81723628382821));
#36367=CARTESIAN_POINT('Ctrl Pts',(-17.8192482499625,7.08972242521831,-2.90349902317069));
#36368=CARTESIAN_POINT('Ctrl Pts',(-17.8123406751945,6.9738347131051,-2.9948061723449));
#36369=CARTESIAN_POINT('Ctrl Pts',(-17.805433730195,6.85795756655736,-3.08610499698111));
#36370=CARTESIAN_POINT('Ctrl Pts',(-17.7985267851956,6.74603118445736,-3.18244710971482));
#36371=CARTESIAN_POINT('Ctrl Pts',(-17.7916198401962,6.63848738561534,-3.28346506457867));
#36372=CARTESIAN_POINT('Ctrl Pts',(-17.7847137708704,6.53095722135077,-3.38447021222218));
#36373=CARTESIAN_POINT('Ctrl Pts',(-17.7778077015447,6.4278087750554,-3.49014978807379));
#36374=CARTESIAN_POINT('Ctrl Pts',(-17.7709016322189,6.32943824184797,-3.60009829050449));
#36375=CARTESIAN_POINT('Ctrl Pts',(-17.763994324437,6.23105006798389,-3.71006650985363));
#36376=CARTESIAN_POINT('Ctrl Pts',(-17.757087016655,6.13744174453664,-3.82430493647222));
#36377=CARTESIAN_POINT('Ctrl Pts',(-17.7501797088731,6.04897067901331,-3.94237323066272));
#36378=CARTESIAN_POINT('Ctrl Pts',(-17.7447864725821,5.97989233816772,-4.03456113210717));
#36379=CARTESIAN_POINT('Ctrl Pts',(-17.739393236291,5.91394518475807,-4.12908318533048));
#36380=CARTESIAN_POINT('Ctrl Pts',(-17.734,5.85128156875001,-4.22571665929507));
#36381=CARTESIAN_POINT('Origin',(-26.8463464956315,10.1295,-7.));
#36382=CARTESIAN_POINT('',(-19.6904980116781,14.1761130084764,-3.89698020567858));
#36383=CARTESIAN_POINT('',(-19.5651698472381,14.1758012177496,-3.89721939943572));
#36384=CARTESIAN_POINT('',(-26.8463464956315,14.1758012177496,-3.89721939943572));
#36385=CARTESIAN_POINT('',(-18.5963464953293,10.1295585775261,-12.0989827703721));
#36386=CARTESIAN_POINT('Ctrl Pts',(-19.5651698472381,14.1758012177496,-3.89721939943573));
#36387=CARTESIAN_POINT('Ctrl Pts',(-19.5580044161035,14.0826682834138,-3.77576578922978));
#36388=CARTESIAN_POINT('Ctrl Pts',(-19.5508389849689,13.9840555505791,-3.65849855785608));
#36389=CARTESIAN_POINT('Ctrl Pts',(-19.5436735538343,13.880367165973,-3.54590149196268));
#36390=CARTESIAN_POINT('Ctrl Pts',(-19.5367389751113,13.7800193638371,-3.43693202414545));
#36391=CARTESIAN_POINT('Ctrl Pts',(-19.5298043963883,13.6749181421213,-3.33233670473415));
#36392=CARTESIAN_POINT('Ctrl Pts',(-19.5228698176653,13.5654689251814,-3.23251827540095));
#36393=CARTESIAN_POINT('Ctrl Pts',(-19.5155889603249,13.4505543548251,-3.1277154066261));
#36394=CARTESIAN_POINT('Ctrl Pts',(-19.5083081029845,13.3308466771977,-3.02817903320695));
#36395=CARTESIAN_POINT('Ctrl Pts',(-19.5010272456441,13.2068564753748,-2.93432931443421));
#36396=CARTESIAN_POINT('Ctrl Pts',(-19.4937463883037,13.0828662735518,-2.84047959566147));
#36397=CARTESIAN_POINT('Ctrl Pts',(-19.4864655309633,12.9545938885293,-2.75231677826634));
#36398=CARTESIAN_POINT('Ctrl Pts',(-19.4791846736229,12.8225874034969,-2.67021002390112));
#36399=CARTESIAN_POINT('Ctrl Pts',(-19.4722525221646,12.6969031736126,-2.59203565096662));
#36400=CARTESIAN_POINT('Ctrl Pts',(-19.4653203707063,12.5677907388499,-2.51932374374965));
#36401=CARTESIAN_POINT('Ctrl Pts',(-19.4583882192479,12.4357445771248,-2.45235918849316));
#36402=CARTESIAN_POINT('Ctrl Pts',(-19.4514574046156,12.3037238797517,-2.38540754697069));
#36403=CARTESIAN_POINT('Ctrl Pts',(-19.4445265899834,12.168770879082,-2.32420119569286));
#36404=CARTESIAN_POINT('Ctrl Pts',(-19.4375957753511,12.0314040081222,-2.26897874197455));
#36405=CARTESIAN_POINT('Ctrl Pts',(-19.4306647326403,11.8940326167085,-2.2137544710018));
#36406=CARTESIAN_POINT('Ctrl Pts',(-19.4237336899295,11.7542475017452,-2.16451461821824));
#36407=CARTESIAN_POINT('Ctrl Pts',(-19.4168026472187,11.6125869069859,-2.12144957735118));
#36408=CARTESIAN_POINT('Ctrl Pts',(-19.4098719853274,11.4709340956326,-2.07838690265165));
#36409=CARTESIAN_POINT('Ctrl Pts',(-19.4029413234362,11.3274063275017,-2.04149845637549));
#36410=CARTESIAN_POINT('Ctrl Pts',(-19.3960106615449,11.1825568421866,-2.01092470620817));
#36411=CARTESIAN_POINT('Ctrl Pts',(-19.3890784541281,11.0376750556868,-1.98034413814746));
#36412=CARTESIAN_POINT('Ctrl Pts',(-19.3821462467112,10.8914712869161,-1.95608114825948));
#36413=CARTESIAN_POINT('Ctrl Pts',(-19.3752140392943,10.7445094240284,-1.93822517210057));
#36414=CARTESIAN_POINT('Ctrl Pts',(-19.3710890357678,10.6570599052498,-1.92759999022186));
#36415=CARTESIAN_POINT('Ctrl Pts',(-19.3669640322412,10.5693421308198,-1.91924244470383));
#36416=CARTESIAN_POINT('Ctrl Pts',(-19.3628390287147,10.481475913415,-1.91316267643876));
#36417=CARTESIAN_POINT('Ctrl Pts',(-19.3559048049855,10.3337708252122,-1.90294244920731));
#36418=CARTESIAN_POINT('Ctrl Pts',(-19.3489705812563,10.1855950223114,-1.89915811409712));
#36419=CARTESIAN_POINT('Ctrl Pts',(-19.3420363575271,10.0375191660747,-1.90182968838914));
#36420=CARTESIAN_POINT('Ctrl Pts',(-19.3351034415158,9.8894712353064,-1.9045007588518));
#36421=CARTESIAN_POINT('Ctrl Pts',(-19.3281705255045,9.74152354381111,-1.9136253036207));
#36422=CARTESIAN_POINT('Ctrl Pts',(-19.3212376094931,9.59424623169765,-1.9291712310986));
#36423=CARTESIAN_POINT('Ctrl Pts',(-19.3143044421616,9.44696358073864,-1.9447177221209));
#36424=CARTESIAN_POINT('Ctrl Pts',(-19.30737127483,9.30035168675085,-1.96668603024645));
#36425=CARTESIAN_POINT('Ctrl Pts',(-19.3004381074985,9.15497560566773,-1.99499218733364));
#36426=CARTESIAN_POINT('Ctrl Pts',(-19.2935053129045,9.00960734022225,-2.02329682263908));
#36427=CARTESIAN_POINT('Ctrl Pts',(-19.2865725183105,8.86547507891971,-2.05793856101137));
#36428=CARTESIAN_POINT('Ctrl Pts',(-19.2796397237165,8.72313373977314,-2.09878230007118));
#36429=CARTESIAN_POINT('Ctrl Pts',(-19.2727053897295,8.58076079443217,-2.13963510828241));
#36430=CARTESIAN_POINT('Ctrl Pts',(-19.2657710557426,8.44017988357931,-2.18669257768057));
#36431=CARTESIAN_POINT('Ctrl Pts',(-19.2588367217556,8.30193143109621,-2.23976953016401));
#36432=CARTESIAN_POINT('Ctrl Pts',(-19.2547222757726,8.21990253098119,-2.27126242542232));
#36433=CARTESIAN_POINT('Ctrl Pts',(-19.2506078297895,8.13869448353687,-2.30487357806509));
#36434=CARTESIAN_POINT('Ctrl Pts',(-19.2464933838065,8.05841702068354,-2.34055622495714));
#36435=CARTESIAN_POINT('Ctrl Pts',(-19.2395600669797,7.92314022125396,-2.40068560741598));
#36436=CARTESIAN_POINT('Ctrl Pts',(-19.232626750153,7.79046037418254,-2.4667205608979));
#36437=CARTESIAN_POINT('Ctrl Pts',(-19.2256934333262,7.66089097296183,-2.53841166493079));
#36438=CARTESIAN_POINT('Ctrl Pts',(-19.218761436208,7.53134623437504,-2.61008912306088));
#36439=CARTESIAN_POINT('Ctrl Pts',(-19.2118294390899,7.40491104954959,-2.68742042376904));
#36440=CARTESIAN_POINT('Ctrl Pts',(-19.2048974419717,7.28207405548853,-2.77011034534907));
#36441=CARTESIAN_POINT('Ctrl Pts',(-19.1979652025665,7.1592327680301,-2.8528031571064));
#36442=CARTESIAN_POINT('Ctrl Pts',(-19.1910329631612,7.03999019913484,-2.94085478267516));
#36443=CARTESIAN_POINT('Ctrl Pts',(-19.184100723756,6.92480620440643,-3.03392654171861));
#36444=CARTESIAN_POINT('Ctrl Pts',(-19.177168859976,6.8096284509534,-3.12699325764406));
#36445=CARTESIAN_POINT('Ctrl Pts',(-19.170236996196,6.69850908820766,-3.22507935421226));
#36446=CARTESIAN_POINT('Ctrl Pts',(-19.163305132416,6.5918750714188,-3.32780571528673));
#36447=CARTESIAN_POINT('Ctrl Pts',(-19.1563717255625,6.48521731727435,-3.43055494384976));
#36448=CARTESIAN_POINT('Ctrl Pts',(-19.1494383187091,6.38304714234844,-3.53794627142115));
#36449=CARTESIAN_POINT('Ctrl Pts',(-19.1425049118557,6.28575524711227,-3.64956312182307));
#36450=CARTESIAN_POINT('Ctrl Pts',(-19.1383858542032,6.22795524574662,-3.71587341509055));
#36451=CARTESIAN_POINT('Ctrl Pts',(-19.1342667965508,6.17187627667052,-3.7836743770029));
#36452=CARTESIAN_POINT('Ctrl Pts',(-19.1301477388983,6.11759365881622,-3.8528729753044));
#36453=CARTESIAN_POINT('Ctrl Pts',(-19.1232141282746,6.02621971662068,-3.96935499056361));
#36454=CARTESIAN_POINT('Ctrl Pts',(-19.1162805176509,5.93990636053414,-4.08983920703717));
#36455=CARTESIAN_POINT('Ctrl Pts',(-19.1093469070272,5.85899051470744,-4.21386473120448));
#36456=CARTESIAN_POINT('Ctrl Pts',(-19.1024146126326,5.77809002939035,-4.3378667112163));
#36457=CARTESIAN_POINT('Ctrl Pts',(-19.095482318238,5.70258519057678,-4.46540838095846));
#36458=CARTESIAN_POINT('Ctrl Pts',(-19.0885500238434,5.63276951068097,-4.5960000194616));
#36459=CARTESIAN_POINT('Ctrl Pts',(-19.0816174848406,5.56295136731649,-4.72659626593262));
#36460=CARTESIAN_POINT('Ctrl Pts',(-19.0746849458378,5.49882294336051,-4.86024240657262));
#36461=CARTESIAN_POINT('Ctrl Pts',(-19.067752406835,5.44063196898206,-4.99642380037644));
#36462=CARTESIAN_POINT('Ctrl Pts',(-19.0608202428625,5.38244414256678,-5.13259782716129));
#36463=CARTESIAN_POINT('Ctrl Pts',(-19.0538880788899,5.33019325204807,-5.27130652831807));
#36464=CARTESIAN_POINT('Ctrl Pts',(-19.0469559149174,5.28407902177485,-5.41201494220643));
#36465=CARTESIAN_POINT('Ctrl Pts',(-19.0400222095796,5.2379545380122,-5.55275464258111));
#36466=CARTESIAN_POINT('Ctrl Pts',(-19.0330885042419,5.19796954390401,-5.69549462988479));
#36467=CARTESIAN_POINT('Ctrl Pts',(-19.0261547989042,5.1642741877754,-5.83968382170268));
#36468=CARTESIAN_POINT('Ctrl Pts',(-19.0220372305995,5.1442642618192,-5.92531031103094));
#36469=CARTESIAN_POINT('Ctrl Pts',(-19.0179196622948,5.12647145780716,-6.01144759299916));
#36470=CARTESIAN_POINT('Ctrl Pts',(-19.0138020939901,5.11091873588374,-6.09797832871864));
#36471=CARTESIAN_POINT('Ctrl Pts',(-19.0068685366575,5.08472956762835,-6.24368709970922));
#36472=CARTESIAN_POINT('Ctrl Pts',(-18.9999349793249,5.06488588872228,-6.39056232944993));
#36473=CARTESIAN_POINT('Ctrl Pts',(-18.9930014219922,5.05146956995229,-6.53803901516524));
#36474=CARTESIAN_POINT('Ctrl Pts',(-18.9860691811566,5.03805579858218,-6.68548769900486));
#36475=CARTESIAN_POINT('Ctrl Pts',(-18.9791369403209,5.03106698243318,-6.83353728193027));
#36476=CARTESIAN_POINT('Ctrl Pts',(-18.9722046994853,5.03053313522663,-6.981617618673));
#36477=CARTESIAN_POINT('Ctrl Pts',(-18.9652722139179,5.02999926917346,-7.12970318315557));
#36478=CARTESIAN_POINT('Ctrl Pts',(-18.9583397283506,5.03592083259744,-7.27781917307014));
#36479=CARTESIAN_POINT('Ctrl Pts',(-18.9514072427832,5.04827571738031,-7.42539486329296));
#36480=CARTESIAN_POINT('Ctrl Pts',(-18.9444751320469,5.06062993414973,-7.57296257427935));
#36481=CARTESIAN_POINT('Ctrl Pts',(-18.9375430213105,5.07941674773549,-7.71998971467166));
#36482=CARTESIAN_POINT('Ctrl Pts',(-18.9306109105741,5.10456211729912,-7.86591008482266));
#36483=CARTESIAN_POINT('Ctrl Pts',(-18.9236772576965,5.12971308078845,-8.01186291692284));
#36484=CARTESIAN_POINT('Ctrl Pts',(-18.9167436048189,5.16122537054672,-8.1567081609133));
#36485=CARTESIAN_POINT('Ctrl Pts',(-18.9098099519412,5.19897359234514,-8.29988858884832));
#36486=CARTESIAN_POINT('Ctrl Pts',(-18.9056921176548,5.22139192287262,-8.38492216144028));
#36487=CARTESIAN_POINT('Ctrl Pts',(-18.9015742833683,5.24600873413897,-8.46936874424748));
#36488=CARTESIAN_POINT('Ctrl Pts',(-18.8974564490819,5.27278935781425,-8.55311388445269));
#36489=CARTESIAN_POINT('Ctrl Pts',(-18.8905228748665,5.31788234331871,-8.69412323655478));
#36490=CARTESIAN_POINT('Ctrl Pts',(-18.883589300651,5.36912832626771,-8.83319175144094));
#36491=CARTESIAN_POINT('Ctrl Pts',(-18.8766557264356,5.42633506454241,-8.96978186352757));
#36492=CARTESIAN_POINT('Ctrl Pts',(-18.8697234691356,5.48353093736216,-9.1063460326265));
#36493=CARTESIAN_POINT('Ctrl Pts',(-18.8627912118356,5.54668517907365,-9.2404324333557));
#36494=CARTESIAN_POINT('Ctrl Pts',(-18.8558589545357,5.61555731959328,-9.37152324003005));
#36495=CARTESIAN_POINT('Ctrl Pts',(-18.8489264532936,5.68443188368328,-9.50261865971326));
#36496=CARTESIAN_POINT('Ctrl Pts',(-18.8419939520516,5.75902459842385,-9.63071798021076));
#36497=CARTESIAN_POINT('Ctrl Pts',(-18.8350614508095,5.83904866843853,-9.75532727121524));
#36498=CARTESIAN_POINT('Ctrl Pts',(-18.8281293248839,5.91906840605573,-9.87992981603726));
#36499=CARTESIAN_POINT('Ctrl Pts',(-18.8211971989583,6.00451873113978,-10.0010424317848));
#36500=CARTESIAN_POINT('Ctrl Pts',(-18.8142650730327,6.09506908079314,-10.1181995058283));
#36501=CARTESIAN_POINT('Ctrl Pts',(-18.8073314058495,6.18563956300298,-10.2353826280473));
#36502=CARTESIAN_POINT('Ctrl Pts',(-18.8003977386663,6.28131213326655,-10.3486081896358));
#36503=CARTESIAN_POINT('Ctrl Pts',(-18.7934640714831,6.3817150551582,-10.4574425529887));
#36504=CARTESIAN_POINT('Ctrl Pts',(-18.7893463157133,6.44134219040977,-10.5220769399308));
#36505=CARTESIAN_POINT('Ctrl Pts',(-18.7852285599435,6.50263691562057,-10.5851632219833));
#36506=CARTESIAN_POINT('Ctrl Pts',(-18.7811108041737,6.56551500754935,-10.646616510354));
#36507=CARTESIAN_POINT('Ctrl Pts',(-18.7741773223733,6.6713892095192,-10.7500916264889));
#36508=CARTESIAN_POINT('Ctrl Pts',(-18.7672438405729,6.78179109135341,-10.8489706372656));
#36509=CARTESIAN_POINT('Ctrl Pts',(-18.7603103587725,6.8962990704977,-10.9428685939891));
#36510=CARTESIAN_POINT('Ctrl Pts',(-18.7533781937436,7.01078530286897,-11.0367487180902));
#36511=CARTESIAN_POINT('Ctrl Pts',(-18.7464460287148,7.12937582121678,-11.1256494659908));
#36512=CARTESIAN_POINT('Ctrl Pts',(-18.739513863686,7.25161567360849,-11.2092259150478));
#36513=CARTESIAN_POINT('Ctrl Pts',(-18.7325814536027,7.37385984722272,-11.2928053185622));
#36514=CARTESIAN_POINT('Ctrl Pts',(-18.7256490435193,7.49975334201189,-11.3710598572636));
#36515=CARTESIAN_POINT('Ctrl Pts',(-18.718716633436,7.62881146378363,-11.4436874152933));
#36516=CARTESIAN_POINT('Ctrl Pts',(-18.7117845978205,7.75786261422604,-11.516311050202));
#36517=CARTESIAN_POINT('Ctrl Pts',(-18.704852562205,7.8900777610185,-11.5833081513277));
#36518=CARTESIAN_POINT('Ctrl Pts',(-18.6979205265895,8.02494679887543,-11.64442211945));
#36519=CARTESIAN_POINT('Ctrl Pts',(-18.6909869476181,8.15984586411981,-11.7055496940518));
#36520=CARTESIAN_POINT('Ctrl Pts',(-18.6840533686468,8.29739969982354,-11.7607913819451));
#36521=CARTESIAN_POINT('Ctrl Pts',(-18.6771197896754,8.43707679425735,-11.8099381173424));
#36522=CARTESIAN_POINT('Ctrl Pts',(-18.6730015795388,8.52003822420948,-11.8391288981399));
#36523=CARTESIAN_POINT('Ctrl Pts',(-18.6688833694022,8.60374831456233,-11.8661704298008));
#36524=CARTESIAN_POINT('Ctrl Pts',(-18.6647651592655,8.68809285583543,-11.8910271359655));
#36525=CARTESIAN_POINT('Ctrl Pts',(-18.6577998241514,8.83074900390097,-11.9330685283489));
#36526=CARTESIAN_POINT('Ctrl Pts',(-18.6508344890373,8.97526829574175,-11.9688711530495));
#36527=CARTESIAN_POINT('Ctrl Pts',(-18.6438691539232,9.12109290423389,-11.9982913209625));
#36528=CARTESIAN_POINT('Ctrl Pts',(-18.6369053501428,9.26688545308524,-12.0277050208312));
#36529=CARTESIAN_POINT('Ctrl Pts',(-18.6299415463624,9.41398242822589,-12.0507390002111));
#36530=CARTESIAN_POINT('Ctrl Pts',(-18.622977742582,9.56181530050721,-12.0673005715037));
#36531=CARTESIAN_POINT('Ctrl Pts',(-18.6160146854246,9.70963232291145,-12.0838603671502));
#36532=CARTESIAN_POINT('Ctrl Pts',(-18.6090516282673,9.85818476303232,-12.0939491026305));
#36533=CARTESIAN_POINT('Ctrl Pts',(-18.60208857111,10.0068979934788,-12.097525845741));
#36534=CARTESIAN_POINT('Ctrl Pts',(-18.6001745459505,10.0477767135858,-12.0985090311648));
#36535=CARTESIAN_POINT('Ctrl Pts',(-18.598260520791,10.0886675622518,-12.099000469371));
#36536=CARTESIAN_POINT('Ctrl Pts',(-18.5963464956315,10.1295585712674,-12.0989999996636));
#36537=CARTESIAN_POINT('Ctrl Pts',(-18.5963464895958,10.1295586962519,-12.098655931404));
#36538=CARTESIAN_POINT('Ctrl Pts',(-18.580370831183,10.4708377603055,-12.0988021573896));
#36539=CARTESIAN_POINT('Ctrl Pts',(-18.5256132911341,11.6404949371434,-11.9829820272798));
#36540=CARTESIAN_POINT('Ctrl Pts',(-18.4320738694491,13.4987506203882,-11.0980785037433));
#36541=CARTESIAN_POINT('Ctrl Pts',(-18.3157282245409,15.0255448975692,-9.04320498956965));
#36542=CARTESIAN_POINT('Ctrl Pts',(-18.1993825796327,15.4123695196911,-6.51259611415262));
#36543=CARTESIAN_POINT('Ctrl Pts',(-18.1158625769727,14.8069605767375,-4.77742165783899));
#36544=CARTESIAN_POINT('Ctrl Pts',(-18.0711244559488,14.2534419862377,-3.99797429297315));
#36545=CARTESIAN_POINT('Ctrl Pts',(-18.0651682165609,14.1759493590362,-3.89710566674782));
#36546=CARTESIAN_POINT('',(-18.7216535051799,10.1294128054764,-12.0989687534116));
#36547=CARTESIAN_POINT('Ctrl Pts',(-18.7216535043684,10.1294128222767,-12.0989999992548));
#36548=CARTESIAN_POINT('Ctrl Pts',(-18.7147113419131,10.2777169024359,-12.0990025348131));
#36549=CARTESIAN_POINT('Ctrl Pts',(-18.7077691794578,10.4260250034406,-12.0925306047745));
#36550=CARTESIAN_POINT('Ctrl Pts',(-18.7008270170026,10.5737648955722,-12.0796092076618));
#36551=CARTESIAN_POINT('Ctrl Pts',(-18.6938850825327,10.7214999358232,-12.0666882348967));
#36552=CARTESIAN_POINT('Ctrl Pts',(-18.6869431480629,10.8686664773571,-12.0473182494839));
#36553=CARTESIAN_POINT('Ctrl Pts',(-18.680001213593,11.0146970824474,-12.021576159457));
#36554=CARTESIAN_POINT('Ctrl Pts',(-18.6730576379768,11.1607622107104,-11.9958279837289));
#36555=CARTESIAN_POINT('Ctrl Pts',(-18.6661140623605,11.3056905422907,-11.9637047507785));
#36556=CARTESIAN_POINT('Ctrl Pts',(-18.6591704867443,11.4489238560583,-11.9253346777721));
#36557=CARTESIAN_POINT('Ctrl Pts',(-18.6552746291148,11.5292883007021,-11.9038062391219));
#36558=CARTESIAN_POINT('Ctrl Pts',(-18.6513787714853,11.6091193479438,-11.8803121893208));
#36559=CARTESIAN_POINT('Ctrl Pts',(-18.6474829138558,11.6883203008384,-11.854882106673));
#36560=CARTESIAN_POINT('Ctrl Pts',(-18.6405493032985,11.8292773417162,-11.8096231916184));
#36561=CARTESIAN_POINT('Ctrl Pts',(-18.6336156927412,11.9682862806913,-11.7582135007032));
#36562=CARTESIAN_POINT('Ctrl Pts',(-18.626682082184,12.1048097739243,-11.7008459129224));
#36563=CARTESIAN_POINT('Ctrl Pts',(-18.6197497878564,12.2413073504607,-11.6434892154165));
#36564=CARTESIAN_POINT('Ctrl Pts',(-18.6128174935289,12.3753201180157,-11.5801770055648));
#36565=CARTESIAN_POINT('Ctrl Pts',(-18.6058851992013,12.5063305296346,-11.5111503669682));
#36566=CARTESIAN_POINT('Ctrl Pts',(-18.5989526602658,12.6373455639937,-11.4421212927467));
#36567=CARTESIAN_POINT('Ctrl Pts',(-18.5920201213302,12.7653577364192,-11.3673775374312));
#36568=CARTESIAN_POINT('Ctrl Pts',(-18.5850875823947,12.8898734499727,-11.2872064816948));
#36569=CARTESIAN_POINT('Ctrl Pts',(-18.5781554184894,13.0143824275872,-11.20703976298));
#36570=CARTESIAN_POINT('Ctrl Pts',(-18.5712232545841,13.1353950473725,-11.121446511085));
#36571=CARTESIAN_POINT('Ctrl Pts',(-18.5642910906788,13.2524460816721,-11.0307578407749));
#36572=CARTESIAN_POINT('Ctrl Pts',(-18.5573573854077,13.3695231422555,-10.9400490058497));
#36573=CARTESIAN_POINT('Ctrl Pts',(-18.5504236801366,13.4826365958723,-10.8442426912284));
#36574=CARTESIAN_POINT('Ctrl Pts',(-18.5434899748654,13.5913532383767,-10.7437111475033));
#36575=CARTESIAN_POINT('Ctrl Pts',(-18.5393724062262,13.6559144246746,-10.6840106676712));
#36576=CARTESIAN_POINT('Ctrl Pts',(-18.5352548375869,13.7189256853204,-10.6226445735402));
#36577=CARTESIAN_POINT('Ctrl Pts',(-18.5311372689476,13.7803022426319,-10.5596971760522));
#36578=CARTESIAN_POINT('Ctrl Pts',(-18.5242037116084,13.8836539816517,-10.453700305551));
#36579=CARTESIAN_POINT('Ctrl Pts',(-18.5172701542692,13.9824041897261,-10.3431810712656));
#36580=CARTESIAN_POINT('Ctrl Pts',(-18.51033659693,14.0761684078321,-10.2285615184816));
#36581=CARTESIAN_POINT('Ctrl Pts',(-18.5034043560879,14.1699148226197,-10.1139637288865));
#36582=CARTESIAN_POINT('Ctrl Pts',(-18.4964721152459,14.2586769270584,-9.99526742983162));
#36583=CARTESIAN_POINT('Ctrl Pts',(-18.4895398744039,14.3421103275237,-9.87292798873217));
#36584=CARTESIAN_POINT('Ctrl Pts',(-18.4826073888305,14.4255466734673,-9.75058422864091));
#36585=CARTESIAN_POINT('Ctrl Pts',(-18.4756749032572,14.5036537499851,-9.62459734036535));
#36586=CARTESIAN_POINT('Ctrl Pts',(-18.4687424176839,14.5761300052532,-9.49545238311256));
#36587=CARTESIAN_POINT('Ctrl Pts',(-18.4618103069418,14.6486023418167,-9.36631440857343));
#36588=CARTESIAN_POINT('Ctrl Pts',(-18.4548781961996,14.7154443053631,-9.23401899548399));
#36589=CARTESIAN_POINT('Ctrl Pts',(-18.4479460854575,14.7763998905137,-9.09907656066754));
#36590=CARTESIAN_POINT('Ctrl Pts',(-18.4410124325745,14.8373690360505,-8.96410410609937));
#36591=CARTESIAN_POINT('Ctrl Pts',(-18.4340787796916,14.8924490504929,-8.82648375455177));
#36592=CARTESIAN_POINT('Ctrl Pts',(-18.4271451268086,14.9414314869883,-8.6867472734616));
#36593=CARTESIAN_POINT('Ctrl Pts',(-18.4230272925522,14.9705217166792,-8.60375903069658));
#36594=CARTESIAN_POINT('Ctrl Pts',(-18.4189094582958,14.9974622098978,-8.52002479361661));
#36595=CARTESIAN_POINT('Ctrl Pts',(-18.4147916240394,15.0222175337942,-8.43565878066583));
#36596=CARTESIAN_POINT('Ctrl Pts',(-18.4078580498408,15.0639003370249,-8.29360400764394));
#36597=CARTESIAN_POINT('Ctrl Pts',(-18.4009244756422,15.099399552533,-8.14970818352137));
#36598=CARTESIAN_POINT('Ctrl Pts',(-18.3939909014436,15.1285731159382,-8.00452425630458));
#36599=CARTESIAN_POINT('Ctrl Pts',(-18.3870586441602,15.1577411383182,-7.85936790432008));
#36600=CARTESIAN_POINT('Ctrl Pts',(-18.3801263868768,15.1805858405798,-7.71292426128418));
#36601=CARTESIAN_POINT('Ctrl Pts',(-18.3731941295934,15.1970161634336,-7.56575695606785));
#36602=CARTESIAN_POINT('Ctrl Pts',(-18.3662616283674,15.2134470644621,-7.41858447210894));
#36603=CARTESIAN_POINT('Ctrl Pts',(-18.3593291271414,15.2234630944089,-7.27068860316924));
#36604=CARTESIAN_POINT('Ctrl Pts',(-18.3523966259154,15.2270249522307,-7.12263915111047));
#36605=CARTESIAN_POINT('Ctrl Pts',(-18.3454645000055,15.2305866172184,-6.9745977142461));
#36606=CARTESIAN_POINT('Ctrl Pts',(-18.3385323740955,15.2276948022499,-6.82640304141275));
#36607=CARTESIAN_POINT('Ctrl Pts',(-18.3316002481857,15.2183623246744,-6.67862601146168));
#36608=CARTESIAN_POINT('Ctrl Pts',(-18.3246665810175,15.2090277721571,-6.53081612541791));
#36609=CARTESIAN_POINT('Ctrl Pts',(-18.3177329138493,15.1932497165721,-6.38342439783593));
#36610=CARTESIAN_POINT('Ctrl Pts',(-18.3107992466811,15.1710929950943,-6.23701830178175));
#36611=CARTESIAN_POINT('Ctrl Pts',(-18.3066814908311,15.1579345946017,-6.15007086922192));
#36612=CARTESIAN_POINT('Ctrl Pts',(-18.3025637349812,15.1425274812019,-6.06347096462069));
#36613=CARTESIAN_POINT('Ctrl Pts',(-18.2984459791312,15.1248938320092,-5.97733609473846));
#36614=CARTESIAN_POINT('Ctrl Pts',(-18.2915125309928,15.0952024183793,-5.83230281083452));
#36615=CARTESIAN_POINT('Ctrl Pts',(-18.2845790828544,15.059185411284,-5.68853843504666));
#36616=CARTESIAN_POINT('Ctrl Pts',(-18.277645634716,15.0169762154728,-5.54659804486579));
#36617=CARTESIAN_POINT('Ctrl Pts',(-18.2703819998395,14.9727569207318,-5.39789812702961));
#36618=CARTESIAN_POINT('Ctrl Pts',(-18.2631183649631,14.9217412775336,-5.25120055839765));
#36619=CARTESIAN_POINT('Ctrl Pts',(-18.2558547300866,14.8641417140795,-5.10712682957934));
#36620=CARTESIAN_POINT('Ctrl Pts',(-18.2489226347855,14.8091712110254,-4.96962916683512));
#36621=CARTESIAN_POINT('Ctrl Pts',(-18.2419905394845,14.7482046250438,-4.83452146236116));
#36622=CARTESIAN_POINT('Ctrl Pts',(-18.2350584441835,14.6814762990125,-4.70232448478292));
#36623=CARTESIAN_POINT('Ctrl Pts',(-18.2281266662119,14.6147510275939,-4.57013355876596));
#36624=CARTESIAN_POINT('Ctrl Pts',(-18.2211948882404,14.5422646938408,-4.44085338759471));
#36625=CARTESIAN_POINT('Ctrl Pts',(-18.2142631102688,14.4642980869847,-4.31498109036941));
#36626=CARTESIAN_POINT('Ctrl Pts',(-18.2073302843237,14.3863196928292,-4.18908976327339));
#36627=CARTESIAN_POINT('Ctrl Pts',(-18.2003974583786,14.3028595456927,-4.06660761962958));
#36628=CARTESIAN_POINT('Ctrl Pts',(-18.1934646324335,14.2142425998208,-3.94800411317289));
#36629=CARTESIAN_POINT('Ctrl Pts',(-18.1924704270217,14.2015344418692,-3.93099571733137));
#36630=CARTESIAN_POINT('Ctrl Pts',(-18.19147622161,14.1887203048187,-3.91406703530483));
#36631=CARTESIAN_POINT('Ctrl Pts',(-18.1904820161982,14.1758012177496,-3.89721939943572));
#36632=CARTESIAN_POINT('Ctrl Pts',(-19.6904980116781,14.1761130084766,-3.89698020567888));
#36633=CARTESIAN_POINT('Ctrl Pts',(-19.6530813654925,13.6895815995602,-3.2628026380609));
#36634=CARTESIAN_POINT('Ctrl Pts',(-19.5768828376708,12.391409734591,-2.20936993870382));
#36635=CARTESIAN_POINT('Ctrl Pts',(-19.4619024282132,9.91265035575874,-1.69885130841003));
#36636=CARTESIAN_POINT('Ctrl Pts',(-19.3455567833049,7.45588094355372,-2.41786028132917));
#36637=CARTESIAN_POINT('Ctrl Pts',(-19.2292111383967,5.62120273326431,-4.20319480177778));
#36638=CARTESIAN_POINT('Ctrl Pts',(-19.1128654934885,4.83646615949574,-6.64003369704514));
#36639=CARTESIAN_POINT('Ctrl Pts',(-18.9965198485804,5.28407824547955,-9.16055201698359));
#36640=CARTESIAN_POINT('Ctrl Pts',(-18.8801742036722,6.85996538611778,-11.1780643879153));
#36641=CARTESIAN_POINT('Ctrl Pts',(-18.7885520913348,8.70047320199483,-12.0007213768745));
#36642=CARTESIAN_POINT('Ctrl Pts',(-18.7357118606335,9.829103193625,-12.0989141769127));
#36643=CARTESIAN_POINT('Ctrl Pts',(-18.7216535115683,10.1294126732152,-12.0987227687564));
#36644=CARTESIAN_POINT('Origin',(-26.8463464956315,10.1295,-7.));
#36645=CARTESIAN_POINT('',(-21.1904791369099,14.1758012177496,-3.89721939943572));
#36646=CARTESIAN_POINT('',(-21.0652864992102,14.1758012177496,-3.89721939943571));
#36647=CARTESIAN_POINT('',(-26.8463464956315,14.1758012177496,-3.89721939943572));
#36648=CARTESIAN_POINT('',(-20.0963464956032,10.1297172757599,-12.0989999953708));
#36649=CARTESIAN_POINT('Ctrl Pts',(-21.0652864992102,14.1758012177496,-3.89721939943571));
#36650=CARTESIAN_POINT('Ctrl Pts',(-21.0585700937333,14.0885055180282,-3.78337806111393));
#36651=CARTESIAN_POINT('Ctrl Pts',(-21.0518536882564,13.996453500271,-3.67329050358813));
#36652=CARTESIAN_POINT('Ctrl Pts',(-21.0451372827796,13.9000084618648,-3.56735277970396));
#36653=CARTESIAN_POINT('Ctrl Pts',(-21.0384166004951,13.8035020101215,-3.46134759782241));
#36654=CARTESIAN_POINT('Ctrl Pts',(-21.0316959182107,13.7025972199478,-3.35949778112184));
#36655=CARTESIAN_POINT('Ctrl Pts',(-21.0249752359262,13.5976933622283,-3.26216161368693));
#36656=CARTESIAN_POINT('Ctrl Pts',(-21.0182444490511,13.4926317808584,-3.16467910067446));
#36657=CARTESIAN_POINT('Ctrl Pts',(-21.0115136621759,13.3835593986938,-3.07172403740939));
#36658=CARTESIAN_POINT('Ctrl Pts',(-21.0047828753008,13.2709083136366,-2.9836142108838));
#36659=CARTESIAN_POINT('Ctrl Pts',(-21.000414602677,13.1977978943015,-2.92643103895467));
#36660=CARTESIAN_POINT('Ctrl Pts',(-20.9960463300532,13.1231807485872,-2.87128781070681));
#36661=CARTESIAN_POINT('Ctrl Pts',(-20.9916780574294,13.0471810287064,-2.81826131678142));
#36662=CARTESIAN_POINT('Ctrl Pts',(-20.9851848243432,12.9342109972609,-2.73943991197112));
#36663=CARTESIAN_POINT('Ctrl Pts',(-20.978691591257,12.8178257484995,-2.66504726072125));
#36664=CARTESIAN_POINT('Ctrl Pts',(-20.9721983581708,12.6984140612851,-2.59540222656693));
#36665=CARTESIAN_POINT('Ctrl Pts',(-20.9657135848688,12.5791579509767,-2.52584793025562));
#36666=CARTESIAN_POINT('Ctrl Pts',(-20.9592288115669,12.4568835846726,-2.46102915145838));
#36667=CARTESIAN_POINT('Ctrl Pts',(-20.9527440382649,12.3320115771828,-2.40122366793344));
#36668=CARTESIAN_POINT('Ctrl Pts',(-20.9462660723299,12.2072706536243,-2.34148096499519));
#36669=CARTESIAN_POINT('Ctrl Pts',(-20.9397881063949,12.0799378707507,-2.28674126299211));
#36670=CARTESIAN_POINT('Ctrl Pts',(-20.93331014046,11.9504610849406,-2.23723801485609));
#36671=CARTESIAN_POINT('Ctrl Pts',(-20.9268373376135,11.8210874951198,-2.18777422195239));
#36672=CARTESIAN_POINT('Ctrl Pts',(-20.920364534767,11.689573674354,-2.14353872349991));
#36673=CARTESIAN_POINT('Ctrl Pts',(-20.9138917319205,11.5563897947138,-2.10471793317875));
#36674=CARTESIAN_POINT('Ctrl Pts',(-20.9074218424767,11.4232658610167,-2.06591461606002));
#36675=CARTESIAN_POINT('Ctrl Pts',(-20.9009519530328,11.2884737466344,-2.03252127528968));
#36676=CARTESIAN_POINT('Ctrl Pts',(-20.894482063589,11.1525008815489,-2.00467516608278));
#36677=CARTESIAN_POINT('Ctrl Pts',(-20.8880136068028,11.0165581255649,-1.97683522296886));
#36678=CARTESIAN_POINT('Ctrl Pts',(-20.8815451500166,10.8794355313577,-1.9545401504312));
#36679=CARTESIAN_POINT('Ctrl Pts',(-20.8750766932304,10.7416323549945,-1.93787643572691));
#36680=CARTESIAN_POINT('Ctrl Pts',(-20.8686081907121,10.603828204361,-1.92121260320993));
#36681=CARTESIAN_POINT('Ctrl Pts',(-20.8621396881938,10.4653438603438,-1.91018025615939));
#36682=CARTESIAN_POINT('Ctrl Pts',(-20.8556711856755,10.3266848256198,-1.90481412070715));
#36683=CARTESIAN_POINT('Ctrl Pts',(-20.8492011591069,10.1879931213035,-1.89944672093442));
#36684=CARTESIAN_POINT('Ctrl Pts',(-20.8427311325383,10.0491270452882,-1.89974820296179));
#36685=CARTESIAN_POINT('Ctrl Pts',(-20.8362611059698,9.91059269125152,-1.90570116795486));
#36686=CARTESIAN_POINT('Ctrl Pts',(-20.8297838192035,9.77190288394293,-1.91166081293638));
#36687=CARTESIAN_POINT('Ctrl Pts',(-20.8233065324372,9.63354594344199,-1.92328458861938));
#36688=CARTESIAN_POINT('Ctrl Pts',(-20.8168292456709,9.49602388099765,-1.94050308759322));
#36689=CARTESIAN_POINT('Ctrl Pts',(-20.8103483111701,9.35842437193014,-1.9577312832992));
#36690=CARTESIAN_POINT('Ctrl Pts',(-20.8038673766692,9.2216610719723,-1.98056040833024));
#36691=CARTESIAN_POINT('Ctrl Pts',(-20.7973864421683,9.08622511032832,-2.00887001726257));
#36692=CARTESIAN_POINT('Ctrl Pts',(-20.7908944963578,8.95055903876625,-2.03722772510241));
#36693=CARTESIAN_POINT('Ctrl Pts',(-20.7844025505473,8.81622519910036,-2.07108441947365));
#36694=CARTESIAN_POINT('Ctrl Pts',(-20.7779106047368,8.68369966808348,-2.11026970066548));
#36695=CARTESIAN_POINT('Ctrl Pts',(-20.7716026590288,8.55493028537938,-2.1483443601778));
#36696=CARTESIAN_POINT('Ctrl Pts',(-20.7652947133209,8.42786837598066,-2.19144945063066));
#36697=CARTESIAN_POINT('Ctrl Pts',(-20.758986767613,8.30292988577589,-2.23938631919967));
#36698=CARTESIAN_POINT('Ctrl Pts',(-20.7522553481606,8.16960385187237,-2.29054135199688));
#36699=CARTESIAN_POINT('Ctrl Pts',(-20.7455239287083,8.0382566326181,-2.34736719785055));
#36700=CARTESIAN_POINT('Ctrl Pts',(-20.7387925092559,7.90939433831116,-2.4096915298711));
#36701=CARTESIAN_POINT('Ctrl Pts',(-20.7320693374223,7.7806899315173,-2.47193949949378));
#36702=CARTESIAN_POINT('Ctrl Pts',(-20.7253461655886,7.65446471705759,-2.53967237964706));
#36703=CARTESIAN_POINT('Ctrl Pts',(-20.718622993755,7.53120645650351,-2.6126691870997));
#36704=CARTESIAN_POINT('Ctrl Pts',(-20.7119066869372,7.40807405468524,-2.68559145767453));
#36705=CARTESIAN_POINT('Ctrl Pts',(-20.7051903801194,7.28790288938902,-2.76376676295887));
#36706=CARTESIAN_POINT('Ctrl Pts',(-20.6984740733016,7.17115757741741,-2.8469275095722));
#36707=CARTESIAN_POINT('Ctrl Pts',(-20.691763254633,7.05450766246991,-2.93002030238408));
#36708=CARTESIAN_POINT('Ctrl Pts',(-20.6850524359643,6.94127832456694,-3.0180902078119));
#36709=CARTESIAN_POINT('Ctrl Pts',(-20.6783416172957,6.83190647329252,-3.11082554613232));
#36710=CARTESIAN_POINT('Ctrl Pts',(-20.6716350376826,6.72260370946926,-3.20350230586892));
#36711=CARTESIAN_POINT('Ctrl Pts',(-20.6649284580695,6.6171538582951,-3.30083838763056));
#36712=CARTESIAN_POINT('Ctrl Pts',(-20.6582218784564,6.51596181868043,-3.40248101990474));
#36713=CARTESIAN_POINT('Ctrl Pts',(-20.651517616954,6.41480475581314,-3.50408851968543));
#36714=CARTESIAN_POINT('Ctrl Pts',(-20.6448133554515,6.31790283410827,-3.60999934380801));
#36715=CARTESIAN_POINT('Ctrl Pts',(-20.638109093949,6.22562508005278,-3.7198229301748));
#36716=CARTESIAN_POINT('Ctrl Pts',(-20.6314059106226,6.13336216605965,-3.82962885476722));
#36717=CARTESIAN_POINT('Ctrl Pts',(-20.6247027272961,6.04572217583957,-3.94334600500746));
#36718=CARTESIAN_POINT('Ctrl Pts',(-20.6179995439696,5.96303463779049,-4.06054981578045));
#36719=CARTESIAN_POINT('Ctrl Pts',(-20.6112961998865,5.88034511671715,-4.17775643735183));
#36720=CARTESIAN_POINT('Ctrl Pts',(-20.6045928558033,5.80260849649827,-4.29844958329638));
#36721=CARTESIAN_POINT('Ctrl Pts',(-20.5978895117201,5.73011159094298,-4.4221748262819));
#36722=CARTESIAN_POINT('Ctrl Pts',(-20.5911822561601,5.65757238262621,-4.54597226434116));
#36723=CARTESIAN_POINT('Ctrl Pts',(-20.5844750006002,5.5902791850645,-4.67280501527352));
#36724=CARTESIAN_POINT('Ctrl Pts',(-20.5777677450402,5.52847358717437,-4.80219269532544));
#36725=CARTESIAN_POINT('Ctrl Pts',(-20.5710584023763,5.46664875716989,-4.93162063708084));
#36726=CARTESIAN_POINT('Ctrl Pts',(-20.5643490597123,5.41031508149065,-5.06360475507181));
#36727=CARTESIAN_POINT('Ctrl Pts',(-20.5576397170484,5.35966624389706,-5.19764405869958));
#36728=CARTESIAN_POINT('Ctrl Pts',(-20.550923952482,5.3089689273521,-5.33181165914898));
#36729=CARTESIAN_POINT('Ctrl Pts',(-20.5442081879156,5.26396744082792,-5.4680380257195));
#36730=CARTESIAN_POINT('Ctrl Pts',(-20.5374924233492,5.22480597472622,-5.60580578166324));
#36731=CARTESIAN_POINT('Ctrl Pts',(-20.533760108165,5.20304182067926,-5.68237080747907));
#36732=CARTESIAN_POINT('Ctrl Pts',(-20.5300277929808,5.18308053177186,-5.75941167581817));
#36733=CARTESIAN_POINT('Ctrl Pts',(-20.5262954777966,5.16494003467883,-5.83683820956401));
#36734=CARTESIAN_POINT('Ctrl Pts',(-20.5195533162237,5.13217051860649,-5.97670372862882));
#36735=CARTESIAN_POINT('Ctrl Pts',(-20.5128111546507,5.10528904643073,-6.11806934857135));
#36736=CARTESIAN_POINT('Ctrl Pts',(-20.5060689930777,5.08442238336995,-6.26041035554948));
#36737=CARTESIAN_POINT('Ctrl Pts',(-20.4993317332857,5.06357089108348,-6.40264787577052));
#36738=CARTESIAN_POINT('Ctrl Pts',(-20.4925944734937,5.04872555025018,-6.54585900974967));
#36739=CARTESIAN_POINT('Ctrl Pts',(-20.4858572137016,5.03996208500966,-6.6895087571673));
#36740=CARTESIAN_POINT('Ctrl Pts',(-20.4791236997966,5.03120349221753,-6.83307863595294));
#36741=CARTESIAN_POINT('Ctrl Pts',(-20.4723901858916,5.02852005962299,-6.97708627789357));
#36742=CARTESIAN_POINT('Ctrl Pts',(-20.4656566719866,5.03193567501759,-7.1209915396491));
#36743=CARTESIAN_POINT('Ctrl Pts',(-20.4589254983211,5.03535010331164,-7.26484678698641));
#36744=CARTESIAN_POINT('Ctrl Pts',(-20.4521943246556,5.04485934699365,-7.40859935977456));
#36745=CARTESIAN_POINT('Ctrl Pts',(-20.4454631509901,5.0604351888477,-7.55170910844169));
#36746=CARTESIAN_POINT('Ctrl Pts',(-20.4387320860167,5.07601077918974,-7.69481654623394));
#36747=CARTESIAN_POINT('Ctrl Pts',(-20.4320010210433,5.09765273928879,-7.83728081633711));
#36748=CARTESIAN_POINT('Ctrl Pts',(-20.4252699560699,5.1252809594022,-7.97856670376547));
#36749=CARTESIAN_POINT('Ctrl Pts',(-20.4201632483428,5.14624186910953,-8.0857571314206));
#36750=CARTESIAN_POINT('Ctrl Pts',(-20.4150565406156,5.17064735025744,-8.19226935385371));
#36751=CARTESIAN_POINT('Ctrl Pts',(-20.4099498328884,5.19844276440152,-8.29787346812079));
#36752=CARTESIAN_POINT('Ctrl Pts',(-20.4026900647831,5.23795711921841,-8.44800177416587));
#36753=CARTESIAN_POINT('Ctrl Pts',(-20.3954302966777,5.28430937275062,-8.59623943939993));
#36754=CARTESIAN_POINT('Ctrl Pts',(-20.3881705285724,5.33729197690511,-8.74199404803374));
#36755=CARTESIAN_POINT('Ctrl Pts',(-20.3809033209466,5.39032887551694,-8.88789802017107));
#36756=CARTESIAN_POINT('Ctrl Pts',(-20.3736361133207,5.45000961080975,-9.03131361418626));
#36757=CARTESIAN_POINT('Ctrl Pts',(-20.3663689056949,5.51607819102709,-9.1716676109601));
#36758=CARTESIAN_POINT('Ctrl Pts',(-20.3590936962913,5.58221951804341,-9.31217614872688));
#36759=CARTESIAN_POINT('Ctrl Pts',(-20.3518184868878,5.65476264327944,-9.44961612005003));
#36760=CARTESIAN_POINT('Ctrl Pts',(-20.3445432774843,5.73340458011022,-9.583436869603));
#36761=CARTESIAN_POINT('Ctrl Pts',(-20.3372657453866,5.81207162428195,-9.7173003429662));
#36762=CARTESIAN_POINT('Ctrl Pts',(-20.329988213289,5.89684123596267,-9.84754207082839));
#36763=CARTESIAN_POINT('Ctrl Pts',(-20.3227106811913,5.98736594979328,-9.97363859776505));
#36764=CARTESIAN_POINT('Ctrl Pts',(-20.3154318373513,6.07790698029596,-10.0997578530329));
#36765=CARTESIAN_POINT('Ctrl Pts',(-20.3081529935112,6.17420503683368,-10.2217302093752));
#36766=CARTESIAN_POINT('Ctrl Pts',(-20.3008741496712,6.2758704453382,-10.3390627809967));
#36767=CARTESIAN_POINT('Ctrl Pts',(-20.2984508291075,6.30971756178363,-10.3781259124288));
#36768=CARTESIAN_POINT('Ctrl Pts',(-20.2960275085439,6.34415926105529,-10.4166750362839));
#36769=CARTESIAN_POINT('Ctrl Pts',(-20.2936041879802,6.3791801760683,-10.4546927820321));
#36770=CARTESIAN_POINT('Ctrl Pts',(-20.2868779809018,6.47638478448219,-10.5602154414733));
#36771=CARTESIAN_POINT('Ctrl Pts',(-20.2801517738235,6.57810999823997,-10.6617018342539));
#36772=CARTESIAN_POINT('Ctrl Pts',(-20.2734255667451,6.68398946099055,-10.7587575241793));
#36773=CARTESIAN_POINT('Ctrl Pts',(-20.2667029434128,6.7898125108012,-10.8557615025012));
#36774=CARTESIAN_POINT('Ctrl Pts',(-20.2599803200806,6.89978512979311,-10.9483392324725));
#36775=CARTESIAN_POINT('Ctrl Pts',(-20.2532576967484,7.01350428426586,-11.0361332608731));
#36776=CARTESIAN_POINT('Ctrl Pts',(-20.2465367266287,7.12719547317678,-11.1239056991614));
#36777=CARTESIAN_POINT('Ctrl Pts',(-20.2398157565091,7.24463107375143,-11.2068965514905));
#36778=CARTESIAN_POINT('Ctrl Pts',(-20.2330947863894,7.36537511122738,-11.2847887461656));
#36779=CARTESIAN_POINT('Ctrl Pts',(-20.2263749847876,7.48609815596555,-11.3626673983881));
#36780=CARTESIAN_POINT('Ctrl Pts',(-20.2196551831858,7.61012818104768,-11.435448961937));
#36781=CARTESIAN_POINT('Ctrl Pts',(-20.212935381584,7.73700061751279,-11.5028599472778));
#36782=CARTESIAN_POINT('Ctrl Pts',(-20.2062137509067,7.86390758762793,-11.570289281343));
#36783=CARTESIAN_POINT('Ctrl Pts',(-20.1994921202293,7.99365819072875,-11.6323449420533));
#36784=CARTESIAN_POINT('Ctrl Pts',(-20.1927704895519,8.12576338186563,-11.6887994801599));
#36785=CARTESIAN_POINT('Ctrl Pts',(-20.1875998407253,8.2273859767871,-11.732227422757));
#36786=CARTESIAN_POINT('Ctrl Pts',(-20.1824291918987,8.33040137579851,-11.7723418012303));
#36787=CARTESIAN_POINT('Ctrl Pts',(-20.1772585430721,8.43457914043762,-11.809058564815));
#36788=CARTESIAN_POINT('Ctrl Pts',(-20.1702026804407,8.57674002221321,-11.8591622266207));
#36789=CARTESIAN_POINT('Ctrl Pts',(-20.1631468178092,8.72111220267323,-11.9029539856882));
#36790=CARTESIAN_POINT('Ctrl Pts',(-20.1560909551778,8.86712880719496,-11.9402651721923));
#36791=CARTESIAN_POINT('Ctrl Pts',(-20.1490348696706,9.01315002398955,-11.9775775372567));
#36792=CARTESIAN_POINT('Ctrl Pts',(-20.1419787841634,9.16081547203784,-12.0084088496475));
#36793=CARTESIAN_POINT('Ctrl Pts',(-20.1349226986562,9.30954582988,-12.0326410719326));
#36794=CARTESIAN_POINT('Ctrl Pts',(-20.1278650246748,9.45830967007435,-12.0568787494039));
#36795=CARTESIAN_POINT('Ctrl Pts',(-20.1208073506934,9.60813859809027,-12.0745143189556));
#36796=CARTESIAN_POINT('Ctrl Pts',(-20.1137496767119,9.75844499148024,-12.085481214266));
#36797=CARTESIAN_POINT('Ctrl Pts',(-20.1079486163518,9.8819894429335,-12.094495461995));
#36798=CARTESIAN_POINT('Ctrl Pts',(-20.1021475559916,10.0058562501456,-12.0990052732534));
#36799=CARTESIAN_POINT('Ctrl Pts',(-20.0963464956315,10.1297172751558,-12.0989999953708));
#36800=CARTESIAN_POINT('Ctrl Pts',(-20.0963464956032,10.1297172757598,-12.0989999953708));
#36801=CARTESIAN_POINT('Ctrl Pts',(-20.089015871315,10.2862367018524,-12.0989933258518));
#36802=CARTESIAN_POINT('Ctrl Pts',(-20.0816852470269,10.4427270477282,-12.0917755131971));
#36803=CARTESIAN_POINT('Ctrl Pts',(-20.0743546227387,10.5985501666255,-12.0773805196369));
#36804=CARTESIAN_POINT('Ctrl Pts',(-20.0698740478804,10.6937913250079,-12.06858210852));
#36805=CARTESIAN_POINT('Ctrl Pts',(-20.0653934730221,10.7887832630484,-12.0571034512937));
#36806=CARTESIAN_POINT('Ctrl Pts',(-20.0609128981638,10.883381113265,-12.0429618546111));
#36807=CARTESIAN_POINT('Ctrl Pts',(-20.0540299000486,11.0287010432615,-12.0212377262588));
#36808=CARTESIAN_POINT('Ctrl Pts',(-20.0471469019333,11.1731216585732,-11.9932218786075));
#36809=CARTESIAN_POINT('Ctrl Pts',(-20.040263903818,11.3160889030018,-11.959012782326));
#36810=CARTESIAN_POINT('Ctrl Pts',(-20.0333828335523,11.4590161039285,-11.924813267624));
#36811=CARTESIAN_POINT('Ctrl Pts',(-20.0265017632867,11.6004904149984,-11.8844240428383));
#36812=CARTESIAN_POINT('Ctrl Pts',(-20.019620693021,11.7399691658932,-11.837994425969));
#36813=CARTESIAN_POINT('Ctrl Pts',(-20.0127398324751,11.8794436657853,-11.7915662241714));
#36814=CARTESIAN_POINT('Ctrl Pts',(-20.0058589719292,12.0169224023365,-11.7390981002918));
#36815=CARTESIAN_POINT('Ctrl Pts',(-19.9989781113832,12.1518786132926,-11.6807890087566));
#36816=CARTESIAN_POINT('Ctrl Pts',(-19.9920977747547,12.2868245485124,-11.6224843569492));
#36817=CARTESIAN_POINT('Ctrl Pts',(-19.9852174381262,12.419248029891,-11.5583397622004));
#36818=CARTESIAN_POINT('Ctrl Pts',(-19.9783371014977,12.5486430535138,-11.4886019969068));
#36819=CARTESIAN_POINT('Ctrl Pts',(-19.9714550222469,12.6780708497566,-11.4188465687294));
#36820=CARTESIAN_POINT('Ctrl Pts',(-19.964572942996,12.8044683557619,-11.3434953008952));
#36821=CARTESIAN_POINT('Ctrl Pts',(-19.9576908637452,12.9273544175526,-11.2628407967201));
#36822=CARTESIAN_POINT('Ctrl Pts',(-19.9533163269153,13.0054659276911,-11.2115734273474));
#36823=CARTESIAN_POINT('Ctrl Pts',(-19.9489417900855,13.0821591944104,-11.1581642466885));
#36824=CARTESIAN_POINT('Ctrl Pts',(-19.9445672532557,13.1573167585015,-11.1026974878654));
#36825=CARTESIAN_POINT('Ctrl Pts',(-19.9376178346047,13.2767125706703,-11.014582621476));
#36826=CARTESIAN_POINT('Ctrl Pts',(-19.9306684159537,13.392276360347,-10.9212397631479));
#36827=CARTESIAN_POINT('Ctrl Pts',(-19.9237189973027,13.5035591632226,-10.8230257340323));
#36828=CARTESIAN_POINT('Ctrl Pts',(-19.9167707096019,13.6148238559054,-10.724827688294));
#36829=CARTESIAN_POINT('Ctrl Pts',(-19.9098224219011,13.7218087066573,-10.6217602701984));
#36830=CARTESIAN_POINT('Ctrl Pts',(-19.9028741342004,13.8240989854157,-10.5142195914549));
#36831=CARTESIAN_POINT('Ctrl Pts',(-19.8959254836163,13.9263946064161,-10.4066732962605));
#36832=CARTESIAN_POINT('Ctrl Pts',(-19.8889768330322,14.0239949372702,-10.2946535083665));
#36833=CARTESIAN_POINT('Ctrl Pts',(-19.8820281824482,14.116522779692,-10.1785925115084));
#36834=CARTESIAN_POINT('Ctrl Pts',(-19.8750798802786,14.209045982645,-10.0625373341027));
#36835=CARTESIAN_POINT('Ctrl Pts',(-19.8681315781091,14.2964970028861,-9.9424416099158));
#36836=CARTESIAN_POINT('Ctrl Pts',(-19.8611832759396,14.3785395224088,-9.81876996879985));
#36837=CARTESIAN_POINT('Ctrl Pts',(-19.8542335347365,14.4605990334123,-9.69507271457101));
#36838=CARTESIAN_POINT('Ctrl Pts',(-19.8472837935334,14.5372476244609,-9.56779833651679));
#36839=CARTESIAN_POINT('Ctrl Pts',(-19.8403340523302,14.6081924776181,-9.43744019227688));
#36840=CARTESIAN_POINT('Ctrl Pts',(-19.8362965710027,14.6494081878925,-9.36170808112577));
#36841=CARTESIAN_POINT('Ctrl Pts',(-19.8322590896751,14.6886996717564,-9.28493568412992));
#36842=CARTESIAN_POINT('Ctrl Pts',(-19.8282216083475,14.7260166271649,-9.20722357186493));
#36843=CARTESIAN_POINT('Ctrl Pts',(-19.8212896270348,14.7900863816857,-9.07379907617413));
#36844=CARTESIAN_POINT('Ctrl Pts',(-19.8143576457221,14.8483539160099,-8.93755987242083));
#36845=CARTESIAN_POINT('Ctrl Pts',(-19.8074256644093,14.9005897744139,-8.79902845015939));
#36846=CARTESIAN_POINT('Ctrl Pts',(-19.800494999141,14.9528157157817,-8.66052332824371));
#36847=CARTESIAN_POINT('Ctrl Pts',(-19.7935643338727,14.9990121492195,-8.51972716550497));
#36848=CARTESIAN_POINT('Ctrl Pts',(-19.7866336686044,15.0389982277045,-8.37718123432116));
#36849=CARTESIAN_POINT('Ctrl Pts',(-19.7797027424108,15.0789858115835,-8.23462993657493));
#36850=CARTESIAN_POINT('Ctrl Pts',(-19.7727718162171,15.1127624801018,-8.09032905625727));
#36851=CARTESIAN_POINT('Ctrl Pts',(-19.7658408900234,15.1401974670158,-7.94483432094795));
#36852=CARTESIAN_POINT('Ctrl Pts',(-19.7589103257021,15.1676310215149,-7.79934718210023));
#36853=CARTESIAN_POINT('Ctrl Pts',(-19.7519797613807,15.1887234966507,-7.65266663834769));
#36854=CARTESIAN_POINT('Ctrl Pts',(-19.7450491970594,15.2033953868547,-7.50535789620315));
#36855=CARTESIAN_POINT('Ctrl Pts',(-19.7381170569175,15.2180706130446,-7.35801566008556));
#36856=CARTESIAN_POINT('Ctrl Pts',(-19.7311849167757,15.2263223045308,-7.21004526955849));
#36857=CARTESIAN_POINT('Ctrl Pts',(-19.7242527766338,15.228122843019,-7.06201697061806));
#36858=CARTESIAN_POINT('Ctrl Pts',(-19.7201271722356,15.2291944182259,-6.97391918426839));
#36859=CARTESIAN_POINT('Ctrl Pts',(-19.7160015678375,15.2279820313568,-6.88580095229293));
#36860=CARTESIAN_POINT('Ctrl Pts',(-19.7118759634393,15.2244886255794,-6.79778252989406));
#36861=CARTESIAN_POINT('Ctrl Pts',(-19.7049446779354,15.2186194751504,-6.64990581745022));
#36862=CARTESIAN_POINT('Ctrl Pts',(-19.6980133924316,15.2063069875029,-6.50225841772228));
#36863=CARTESIAN_POINT('Ctrl Pts',(-19.6910821069277,15.1875929083198,-6.35540933081153));
#36864=CARTESIAN_POINT('Ctrl Pts',(-19.6841521797915,15.1688824966527,-6.20858902284129));
#36865=CARTESIAN_POINT('Ctrl Pts',(-19.6772222526554,15.1437730382402,-6.06256704375094));
#36866=CARTESIAN_POINT('Ctrl Pts',(-19.6702923255192,15.1123580259662,-5.91790624571443));
#36867=CARTESIAN_POINT('Ctrl Pts',(-19.6633621941248,15.080942087741,-5.77324118382958));
#36868=CARTESIAN_POINT('Ctrl Pts',(-19.6564320627304,15.0432202905388,-5.62993770751543));
#36869=CARTESIAN_POINT('Ctrl Pts',(-19.649501931336,14.9993371489926,-5.48854800198896));
#36870=CARTESIAN_POINT('Ctrl Pts',(-19.6425721921158,14.9554564907815,-5.34716629766766));
#36871=CARTESIAN_POINT('Ctrl Pts',(-19.6356424528957,14.9054152848105,-5.20769846335097));
#36872=CARTESIAN_POINT('Ctrl Pts',(-19.6287127136755,14.8494077822419,-5.07068107169067));
#36873=CARTESIAN_POINT('Ctrl Pts',(-19.6217814385138,14.793387865894,-4.93363331081956));
#36874=CARTESIAN_POINT('Ctrl Pts',(-19.614850163352,14.7313991358925,-4.79903738439233));
#36875=CARTESIAN_POINT('Ctrl Pts',(-19.6079188881903,14.6636840544645,-4.66741003169438));
#36876=CARTESIAN_POINT('Ctrl Pts',(-19.6037893649706,14.6233406840806,-4.58898893360879));
#36877=CARTESIAN_POINT('Ctrl Pts',(-19.5996598417508,14.5809656252748,-4.5116211384534));
#36878=CARTESIAN_POINT('Ctrl Pts',(-19.5955303185311,14.5366179506424,-4.43541185194857));
#36879=CARTESIAN_POINT('Ctrl Pts',(-19.5885944518774,14.4621324613293,-4.30741222079398));
#36880=CARTESIAN_POINT('Ctrl Pts',(-19.5816585852237,14.3820543577257,-4.18263838139734));
#36881=CARTESIAN_POINT('Ctrl Pts',(-19.5747227185701,14.296687716155,-4.06157396922663));
#36882=CARTESIAN_POINT('Ctrl Pts',(-19.5715384281261,14.2574954717591,-4.00599270303001));
#36883=CARTESIAN_POINT('Ctrl Pts',(-19.5683541376821,14.2171891408564,-3.95119292358269));
#36884=CARTESIAN_POINT('Ctrl Pts',(-19.5651698472381,14.1758012177496,-3.89721939943573));
#36885=CARTESIAN_POINT('',(-20.2216535043684,10.1252586289357,-12.098998236004));
#36886=CARTESIAN_POINT('Ctrl Pts',(-20.2216531624029,10.1252652855325,-12.0997546424994));
#36887=CARTESIAN_POINT('Ctrl Pts',(-20.1623123258533,11.389567257658,-12.087821313962));
#36888=CARTESIAN_POINT('Ctrl Pts',(-20.0641896076676,13.4904584433699,-11.2892797426427));
#36889=CARTESIAN_POINT('Ctrl Pts',(-19.9272850078459,15.1309521650029,-8.75245213992368));
#36890=CARTESIAN_POINT('Ctrl Pts',(-19.8109393629377,15.377488382025,-6.21192549167328));
#36891=CARTESIAN_POINT('Ctrl Pts',(-19.7320103642151,14.7099924706043,-4.60515278330599));
#36892=CARTESIAN_POINT('Ctrl Pts',(-19.6918632471286,14.1938652656919,-3.92011968463998));
#36893=CARTESIAN_POINT('Ctrl Pts',(-19.6904980116781,14.1761130084766,-3.89698020567888));
#36894=CARTESIAN_POINT('Ctrl Pts',(-21.1904791369099,14.1758012177496,-3.89721939943572));
#36895=CARTESIAN_POINT('Ctrl Pts',(-21.1834164152794,14.084049569575,-3.7775671089476));
#36896=CARTESIAN_POINT('Ctrl Pts',(-21.1763536936489,13.9869830080975,-3.66198180115258));
#36897=CARTESIAN_POINT('Ctrl Pts',(-21.1692909720185,13.8849805995519,-3.55091802556254));
#36898=CARTESIAN_POINT('Ctrl Pts',(-21.1622286881234,13.7829845129405,-3.43986113351475));
#36899=CARTESIAN_POINT('Ctrl Pts',(-21.1551664042283,13.6760533941024,-3.33332543922702));
#36900=CARTESIAN_POINT('Ctrl Pts',(-21.1481041203332,13.5646048872596,-3.23173044839874));
#36901=CARTESIAN_POINT('Ctrl Pts',(-21.1410431083921,13.453176452872,-3.13015375535622));
#36902=CARTESIAN_POINT('Ctrl Pts',(-21.133982096451,13.3372324800264,-3.03351619308533));
#36903=CARTESIAN_POINT('Ctrl Pts',(-21.12692108451,13.217225829596,-2.94219884651238));
#36904=CARTESIAN_POINT('Ctrl Pts',(-21.1198610202629,13.0972352858636,-2.85089375610116));
#36905=CARTESIAN_POINT('Ctrl Pts',(-21.1128009560159,12.9731833943003,-2.76490764052895));
#36906=CARTESIAN_POINT('Ctrl Pts',(-21.1057408917689,12.8455548055735,-2.68458028772159));
#36907=CARTESIAN_POINT('Ctrl Pts',(-21.1007410801552,12.7551705147481,-2.62769388875879));
#36908=CARTESIAN_POINT('Ctrl Pts',(-21.0957412685416,12.6629931066556,-2.57364462842989));
#36909=CARTESIAN_POINT('Ctrl Pts',(-21.0907414569279,12.5692033929549,-2.52253996618568));
#36910=CARTESIAN_POINT('Ctrl Pts',(-21.0840199577374,12.4431171454252,-2.45383738847869));
#36911=CARTESIAN_POINT('Ctrl Pts',(-21.0772984585468,12.314077704637,-2.39043779766261));
#36912=CARTESIAN_POINT('Ctrl Pts',(-21.0705769593563,12.1825638082227,-2.33258851188732));
#36913=CARTESIAN_POINT('Ctrl Pts',(-21.0638571099993,12.0510821927081,-2.27475342557725));
#36914=CARTESIAN_POINT('Ctrl Pts',(-21.0571372606424,11.917127668362,-2.22246607754469));
#36915=CARTESIAN_POINT('Ctrl Pts',(-21.0504174112854,11.7812007609424,-2.17592645202187));
#36916=CARTESIAN_POINT('Ctrl Pts',(-21.0436962436786,11.6452471883978,-2.12937769670307));
#36917=CARTESIAN_POINT('Ctrl Pts',(-21.0369750760718,11.5073208059466,-2.08857904163402));
#36918=CARTESIAN_POINT('Ctrl Pts',(-21.030253908465,11.3679394888552,-2.05368130500631));
#36919=CARTESIAN_POINT('Ctrl Pts',(-21.0235322550113,11.2285480964326,-2.01878104575747));
#36920=CARTESIAN_POINT('Ctrl Pts',(-21.0168106015575,11.0877019181292,-1.98978263908411));
#36921=CARTESIAN_POINT('Ctrl Pts',(-21.0100889481037,10.9459306945814,-1.96678612406095));
#36922=CARTESIAN_POINT('Ctrl Pts',(-21.00336283355,10.8040653787671,-1.94377434646078));
#36923=CARTESIAN_POINT('Ctrl Pts',(-20.9966367189962,10.6612741552293,-1.92677247459321));
#36924=CARTESIAN_POINT('Ctrl Pts',(-20.9899106044424,10.5180941451527,-1.91582891806805));
#36925=CARTESIAN_POINT('Ctrl Pts',(-20.9847390069682,10.4080054197,-1.90741459969268));
#36926=CARTESIAN_POINT('Ctrl Pts',(-20.9795674094939,10.297687025457,-1.90258079609333));
#36927=CARTESIAN_POINT('Ctrl Pts',(-20.9743958120197,10.1873835904047,-1.90132855638237));
#36928=CARTESIAN_POINT('Ctrl Pts',(-20.9671170684873,10.0321374757399,-1.89956609676666));
#36929=CARTESIAN_POINT('Ctrl Pts',(-20.959838324955,9.87682543926592,-1.90489862489669));
#36930=CARTESIAN_POINT('Ctrl Pts',(-20.9525595814226,9.7220753784726,-1.91730325734721));
#36931=CARTESIAN_POINT('Ctrl Pts',(-20.9452817167969,9.56734400371569,-1.92970639194104));
#36932=CARTESIAN_POINT('Ctrl Pts',(-20.9380038521713,9.41317472155407,-1.94917990409636));
#36933=CARTESIAN_POINT('Ctrl Pts',(-20.9307259875456,9.26019127590926,-1.97564896307795));
#36934=CARTESIAN_POINT('Ctrl Pts',(-20.9234524716548,9.10729924230271,-2.00210220603041));
#36935=CARTESIAN_POINT('Ctrl Pts',(-20.9161789557639,8.95559187901386,-2.03554260156708));
#36936=CARTESIAN_POINT('Ctrl Pts',(-20.9089054398731,8.80568411965762,-2.07584397942619));
#36937=CARTESIAN_POINT('Ctrl Pts',(-20.9016367742746,8.65587632522299,-2.11611848259851));
#36938=CARTESIAN_POINT('Ctrl Pts',(-20.894368108676,8.50786598368629,-2.16324476993341));
#36939=CARTESIAN_POINT('Ctrl Pts',(-20.8870994430774,8.36225537649466,-2.21704615946469));
#36940=CARTESIAN_POINT('Ctrl Pts',(-20.8798397779555,8.21682507266881,-2.27078092904428));
#36941=CARTESIAN_POINT('Ctrl Pts',(-20.8725801128336,8.07378880792323,-2.33117421095855));
#36942=CARTESIAN_POINT('Ctrl Pts',(-20.8653204477117,7.93373154482647,-2.39800022911074));
#36943=CARTESIAN_POINT('Ctrl Pts',(-20.862897020845,7.88697752400415,-2.42030814071116));
#36944=CARTESIAN_POINT('Ctrl Pts',(-20.8604735939782,7.84055533141693,-2.44333248635513));
#36945=CARTESIAN_POINT('Ctrl Pts',(-20.8580501671115,7.79448628016983,-2.46706365275169));
#36946=CARTESIAN_POINT('Ctrl Pts',(-20.8513195102469,7.6665373082926,-2.53297294021673));
#36947=CARTESIAN_POINT('Ctrl Pts',(-20.8445888533824,7.54135727855362,-2.6043155917558));
#36948=CARTESIAN_POINT('Ctrl Pts',(-20.8378581965178,7.41941799831926,-2.68082686800284));
#36949=CARTESIAN_POINT('Ctrl Pts',(-20.8311277589209,7.29748269055658,-2.75733565170707));
#36950=CARTESIAN_POINT('Ctrl Pts',(-20.824397321324,7.17878823114962,-2.83901252941112));
#36951=CARTESIAN_POINT('Ctrl Pts',(-20.8176668837272,7.06377874695439,-2.92554860151401));
#36952=CARTESIAN_POINT('Ctrl Pts',(-20.8109330039709,6.94871044325873,-3.01212893091069));
#36953=CARTESIAN_POINT('Ctrl Pts',(-20.8041991242146,6.83733117429048,-3.10357320184736));
#36954=CARTESIAN_POINT('Ctrl Pts',(-20.7974652444583,6.73005358099377,-3.19953094417206));
#36955=CARTESIAN_POINT('Ctrl Pts',(-20.7907296988947,6.62274944968287,-3.29551242423964));
#36956=CARTESIAN_POINT('Ctrl Pts',(-20.7839941533312,6.51954928410615,-3.3960093515451));
#36957=CARTESIAN_POINT('Ctrl Pts',(-20.7772586077676,6.42082972916417,-3.50063351130258));
#36958=CARTESIAN_POINT('Ctrl Pts',(-20.7705168109826,6.32201855316575,-3.60535477214659));
#36959=CARTESIAN_POINT('Ctrl Pts',(-20.7637750141976,6.22769654299804,-3.7142106479578));
#36960=CARTESIAN_POINT('Ctrl Pts',(-20.7570332174125,6.13820130284807,-3.82677833895687));
#36961=CARTESIAN_POINT('Ctrl Pts',(-20.7519236523428,6.07037342734832,-3.91209267877634));
#36962=CARTESIAN_POINT('Ctrl Pts',(-20.746814087273,6.00531726134624,-3.99953837678175));
#36963=CARTESIAN_POINT('Ctrl Pts',(-20.7417045222033,5.9431632940884,-4.08892013425649));
#36964=CARTESIAN_POINT('Ctrl Pts',(-20.7349885840485,5.86146902178138,-4.20640221877302));
#36965=CARTESIAN_POINT('Ctrl Pts',(-20.7282726458937,5.78464992982721,-4.32743176090145));
#36966=CARTESIAN_POINT('Ctrl Pts',(-20.7215567077389,5.7130174542218,-4.45157246074436));
#36967=CARTESIAN_POINT('Ctrl Pts',(-20.7148461284493,5.64144213649508,-4.57561410469117));
#36968=CARTESIAN_POINT('Ctrl Pts',(-20.7081355491596,5.57504537611949,-4.7027616427771));
#36969=CARTESIAN_POINT('Ctrl Pts',(-20.70142496987,5.51409512437858,-4.83255015419271));
#36970=CARTESIAN_POINT('Ctrl Pts',(-20.6947183775871,5.45318108546705,-4.96226155338837));
#36971=CARTESIAN_POINT('Ctrl Pts',(-20.6880117853042,5.39770726562999,-5.09461046626493));
#36972=CARTESIAN_POINT('Ctrl Pts',(-20.6813051930213,5.34789546567046,-5.22910783013783));
#36973=CARTESIAN_POINT('Ctrl Pts',(-20.6746012193564,5.29810311494418,-5.36355267893188));
#36974=CARTESIAN_POINT('Ctrl Pts',(-20.6678972456915,5.25396850735601,-5.50014396102834));
#36975=CARTESIAN_POINT('Ctrl Pts',(-20.6611932720266,5.21566509698604,-5.63837319873549));
#36976=CARTESIAN_POINT('Ctrl Pts',(-20.6544892305015,5.17736129889407,-5.77660383565271));
#36977=CARTESIAN_POINT('Ctrl Pts',(-20.6477851889764,5.14488892341433,-5.91647210752719));
#36978=CARTESIAN_POINT('Ctrl Pts',(-20.6410811474513,5.11837144179936,-6.05745473679721));
#36979=CARTESIAN_POINT('Ctrl Pts',(-20.6343767553807,5.09185257362039,-6.19844473786225));
#36980=CARTESIAN_POINT('Ctrl Pts',(-20.6276723633102,5.07128928850261,-6.34054884896783));
#36981=CARTESIAN_POINT('Ctrl Pts',(-20.6209679712396,5.05675377886097,-6.48323431236225));
#36982=CARTESIAN_POINT('Ctrl Pts',(-20.6142619894755,5.0422148226719,-6.62595360822839));
#36983=CARTESIAN_POINT('Ctrl Pts',(-20.6075560077115,5.03370652666764,-6.76925416302939));
#36984=CARTESIAN_POINT('Ctrl Pts',(-20.6008500259474,5.03124911809655,-6.91259894067772));
#36985=CARTESIAN_POINT('Ctrl Pts',(-20.5941412144946,5.02879067258535,-7.05600420478707));
#36986=CARTESIAN_POINT('Ctrl Pts',(-20.5874324030418,5.03238820704158,-7.19945335934861));
#36987=CARTESIAN_POINT('Ctrl Pts',(-20.5807235915889,5.04200983658002,-7.34241033440146));
#36988=CARTESIAN_POINT('Ctrl Pts',(-20.5740068318481,5.051642865378,-7.48553667823489));
#36989=CARTESIAN_POINT('Ctrl Pts',(-20.5672900721072,5.06731422089053,-7.62816930839583));
#36990=CARTESIAN_POINT('Ctrl Pts',(-20.5605733123664,5.0889401403371,-7.76977743611718));
#36991=CARTESIAN_POINT('Ctrl Pts',(-20.5538521696222,5.11058017171852,-7.91147796983666));
#36992=CARTESIAN_POINT('Ctrl Pts',(-20.5471310268781,5.13818244351978,-8.05215230563819));
#36993=CARTESIAN_POINT('Ctrl Pts',(-20.540409884134,5.1716123485166,-8.1912812578348));
#36994=CARTESIAN_POINT('Ctrl Pts',(-20.5336788198585,5.2050916016471,-8.3306155876456));
#36995=CARTESIAN_POINT('Ctrl Pts',(-20.526947755583,5.24441557450129,-8.46839962056696));
#36996=CARTESIAN_POINT('Ctrl Pts',(-20.5202166913075,5.28939995726636,-8.60412985020847));
#36997=CARTESIAN_POINT('Ctrl Pts',(-20.5164822050006,5.31435790664599,-8.6794348336817));
#36998=CARTESIAN_POINT('Ctrl Pts',(-20.5127477186938,5.34105737182245,-8.75410796890097));
#36999=CARTESIAN_POINT('Ctrl Pts',(-20.5090132323869,5.36946062600318,-8.82806623457683));
#37000=CARTESIAN_POINT('Ctrl Pts',(-20.502520006881,5.41884592811497,-8.95665893986427));
#37001=CARTESIAN_POINT('Ctrl Pts',(-20.4960267813751,5.47354175068292,-9.08349785559962));
#37002=CARTESIAN_POINT('Ctrl Pts',(-20.4895335558692,5.53340481851077,-9.20810101279165));
#37003=CARTESIAN_POINT('Ctrl Pts',(-20.4830487901846,5.59318989261193,-9.33254182841081));
#37004=CARTESIAN_POINT('Ctrl Pts',(-20.4765640245,5.65812865411813,-9.45475232040486));
#37005=CARTESIAN_POINT('Ctrl Pts',(-20.4700792588154,5.72802843516658,-9.57426670412428));
#37006=CARTESIAN_POINT('Ctrl Pts',(-20.4636013005293,5.79785483875086,-9.6936556273304));
#37007=CARTESIAN_POINT('Ctrl Pts',(-20.4571233422431,5.87263170391494,-9.81035372750212));
#37008=CARTESIAN_POINT('Ctrl Pts',(-20.450645383957,5.95211895982359,-9.92391666180394));
#37009=CARTESIAN_POINT('Ctrl Pts',(-20.4441725887856,6.03154286215628,-10.0373890832568));
#37010=CARTESIAN_POINT('Ctrl Pts',(-20.4376997936142,6.11566945835049,-10.1477309823946));
#37011=CARTESIAN_POINT('Ctrl Pts',(-20.4312269984427,6.20421383286382,-10.2545244669674));
#37012=CARTESIAN_POINT('Ctrl Pts',(-20.4247571166935,6.29271835332039,-10.3612698835108));
#37013=CARTESIAN_POINT('Ctrl Pts',(-20.4182872349443,6.38563644465789,-10.4644697516912));
#37014=CARTESIAN_POINT('Ctrl Pts',(-20.4118173531951,6.48264134772176,-10.5637372195917));
#37015=CARTESIAN_POINT('Ctrl Pts',(-20.4053489041175,6.57962477030434,-10.6629827059953));
#37016=CARTESIAN_POINT('Ctrl Pts',(-20.39888045504,6.68069292567982,-10.7582972360804));
#37017=CARTESIAN_POINT('Ctrl Pts',(-20.3924120059624,6.78548080763127,-10.8493293754977));
#37018=CARTESIAN_POINT('Ctrl Pts',(-20.3859435111625,6.89026943027771,-10.9403621583773));
#37019=CARTESIAN_POINT('Ctrl Pts',(-20.3794750163626,6.99877752904281,-11.0271122270101));
#37020=CARTESIAN_POINT('Ctrl Pts',(-20.3730065215627,7.11060591490089,-11.1092675141628));
#37021=CARTESIAN_POINT('Ctrl Pts',(-20.3665365027179,7.22246064869354,-11.1914421579583));
#37022=CARTESIAN_POINT('Ctrl Pts',(-20.3600664838731,7.33763690188177,-11.2690196300627));
#37023=CARTESIAN_POINT('Ctrl Pts',(-20.3535964650283,7.45570578264319,-11.3417307013712));
#37024=CARTESIAN_POINT('Ctrl Pts',(-20.347119185956,7.57390715249828,-11.4145233642377));
#37025=CARTESIAN_POINT('Ctrl Pts',(-20.3406419068838,7.69500729020921,-11.4824385099356));
#37026=CARTESIAN_POINT('Ctrl Pts',(-20.3341646278115,7.81855153687926,-11.5452522703146));
#37027=CARTESIAN_POINT('Ctrl Pts',(-20.3276837010034,7.9421653585622,-11.6081014048069));
#37028=CARTESIAN_POINT('Ctrl Pts',(-20.3212027741953,8.06822566499679,-11.6658432682261));
#37029=CARTESIAN_POINT('Ctrl Pts',(-20.3147218473872,8.19625820555243,-11.7183023604048));
#37030=CARTESIAN_POINT('Ctrl Pts',(-20.3082299091909,8.3245082791934,-11.7708505829571));
#37031=CARTESIAN_POINT('Ctrl Pts',(-20.3017379709947,8.45473690394363,-11.818097967878));
#37032=CARTESIAN_POINT('Ctrl Pts',(-20.2952460327984,8.58645429869657,-11.8599188227468));
#37033=CARTESIAN_POINT('Ctrl Pts',(-20.2889380027224,8.71444031188824,-11.9005549474817));
#37034=CARTESIAN_POINT('Ctrl Pts',(-20.2826299726465,8.84383154608124,-11.9360678348261));
#37035=CARTESIAN_POINT('Ctrl Pts',(-20.2763219425705,8.97417216558045,-11.9663888888221));
#37036=CARTESIAN_POINT('Ctrl Pts',(-20.2664274954747,9.17861766576668,-12.0139489132734));
#37037=CARTESIAN_POINT('Ctrl Pts',(-20.2565330483789,9.38595698020578,-12.0488706803317));
#37038=CARTESIAN_POINT('Ctrl Pts',(-20.2466386012831,9.59491891455191,-12.0708997291488));
#37039=CARTESIAN_POINT('Ctrl Pts',(-20.2383102356448,9.77080659951878,-12.0894420460094));
#37040=CARTESIAN_POINT('Ctrl Pts',(-20.2299818700066,9.94784426009558,-12.0988506618854));
#37041=CARTESIAN_POINT('Ctrl Pts',(-20.2216535043684,10.1252586289357,-12.098998236004));
#37042=CARTESIAN_POINT('Origin',(-26.8463464956315,10.1295,-7.));
#37043=CARTESIAN_POINT('',(-22.6904763727661,14.1758012177496,-3.89721939943571));
#37044=CARTESIAN_POINT('',(-22.5651720736883,14.1754919335057,-3.89745664672315));
#37045=CARTESIAN_POINT('',(-26.8463464956315,14.1758012177496,-3.89721939943572));
#37046=CARTESIAN_POINT('',(-23.2216535038438,10.1296134641623,-12.0989489123299));
#37047=CARTESIAN_POINT('Ctrl Pts',(-23.2216535036443,10.1296134695606,-12.0989999987375));
#37048=CARTESIAN_POINT('Ctrl Pts',(-23.2144616176573,10.2832380933687,-12.0989965800831));
#37049=CARTESIAN_POINT('Ctrl Pts',(-23.2072697316703,10.4368320308009,-12.092046129591));
#37050=CARTESIAN_POINT('Ctrl Pts',(-23.2000778456833,10.589781612833,-12.0781829266863));
#37051=CARTESIAN_POINT('Ctrl Pts',(-23.1950395855473,10.6969301109268,-12.0684710899472));
#37052=CARTESIAN_POINT('Ctrl Pts',(-23.1900013254114,10.80376240697,-12.0553677903385));
#37053=CARTESIAN_POINT('Ctrl Pts',(-23.1849630652754,10.9100690396704,-12.0388999766128));
#37054=CARTESIAN_POINT('Ctrl Pts',(-23.1780322210911,11.0563089493057,-12.016246154081));
#37055=CARTESIAN_POINT('Ctrl Pts',(-23.1711013769068,11.2015880256627,-11.9872177039362));
#37056=CARTESIAN_POINT('Ctrl Pts',(-23.1641705327225,11.3453457830432,-11.9519208426484));
#37057=CARTESIAN_POINT('Ctrl Pts',(-23.1572410393046,11.4890755231802,-11.9166308604382));
#37058=CARTESIAN_POINT('Ctrl Pts',(-23.1503115458867,11.6312842144825,-11.875074983332));
#37059=CARTESIAN_POINT('Ctrl Pts',(-23.1433820524688,11.7714233688928,-11.8274101390584));
#37060=CARTESIAN_POINT('Ctrl Pts',(-23.1364523390414,11.9115669726828,-11.779743781439));
#37061=CARTESIAN_POINT('Ctrl Pts',(-23.129522625614,12.0496405935019,-11.725968171853));
#37062=CARTESIAN_POINT('Ctrl Pts',(-23.1225929121865,12.1851121473728,-11.666289714492));
#37063=CARTESIAN_POINT('Ctrl Pts',(-23.1156635809782,12.3205762291,-11.6066145487888));
#37064=CARTESIAN_POINT('Ctrl Pts',(-23.1087342497699,12.453438228391,-11.5410373210932));
#37065=CARTESIAN_POINT('Ctrl Pts',(-23.1018049185616,12.5831872350453,-11.4698120712817));
#37066=CARTESIAN_POINT('Ctrl Pts',(-23.0948740323597,12.7129653583441,-11.3985708379931));
#37067=CARTESIAN_POINT('Ctrl Pts',(-23.0879431461578,12.8396288027836,-11.3216792094331));
#37068=CARTESIAN_POINT('Ctrl Pts',(-23.0810122599559,12.9626918508012,-11.2394368654992));
#37069=CARTESIAN_POINT('Ctrl Pts',(-23.0768806467596,13.0360517211474,-11.1904108760966));
#37070=CARTESIAN_POINT('Ctrl Pts',(-23.0727490335634,13.1081326835169,-11.1394843440002));
#37071=CARTESIAN_POINT('Ctrl Pts',(-23.0686174203672,13.1788367906057,-11.0867280478958));
#37072=CARTESIAN_POINT('Ctrl Pts',(-23.0616832477982,13.2975009676742,-10.9981860562044));
#37073=CARTESIAN_POINT('Ctrl Pts',(-23.0547490752291,13.4123264715572,-10.9044570184215));
#37074=CARTESIAN_POINT('Ctrl Pts',(-23.0478149026601,13.5228675281008,-10.8058977678376));
#37075=CARTESIAN_POINT('Ctrl Pts',(-23.0408820410097,13.6333876866445,-10.7073571500701));
#37076=CARTESIAN_POINT('Ctrl Pts',(-23.0339491793593,13.7396247673742,-10.6039883612046));
#37077=CARTESIAN_POINT('Ctrl Pts',(-23.027016317709,13.8411673613832,-10.4961874089417));
#37078=CARTESIAN_POINT('Ctrl Pts',(-23.0200832090312,13.9427135734955,-10.3883826155816));
#37079=CARTESIAN_POINT('Ctrl Pts',(-23.0131501003533,14.0395647351762,-10.2761455810761));
#37080=CARTESIAN_POINT('Ctrl Pts',(-23.0062169916755,14.131347111674,-10.1599083364532));
#37081=CARTESIAN_POINT('Ctrl Pts',(-22.9992842580324,14.2231245233599,-10.0436773794868));
#37082=CARTESIAN_POINT('Ctrl Pts',(-22.9923515243894,14.3098334944501,-9.9234469053268));
#37083=CARTESIAN_POINT('Ctrl Pts',(-22.9854187907463,14.3911413124602,-9.79968111111478));
#37084=CARTESIAN_POINT('Ctrl Pts',(-22.9784845207415,14.4724671490789,-9.67588788919075));
#37085=CARTESIAN_POINT('Ctrl Pts',(-22.9715502507368,14.5483892594452,-9.54855805804282));
#37086=CARTESIAN_POINT('Ctrl Pts',(-22.9646159807321,14.6186185668019,-9.41818433813362));
#37087=CARTESIAN_POINT('Ctrl Pts',(-22.960501245641,14.6602920227245,-9.34082171454237));
#37088=CARTESIAN_POINT('Ctrl Pts',(-22.95638651055,14.6999618159018,-9.26238781469777));
#37089=CARTESIAN_POINT('Ctrl Pts',(-22.952271775459,14.7375752110852,-9.18298965846895));
#37090=CARTESIAN_POINT('Ctrl Pts',(-22.9453381247487,14.800956726167,-9.04919755031274));
#37091=CARTESIAN_POINT('Ctrl Pts',(-22.9384044740384,14.8585183931822,-8.91262019456305));
#37092=CARTESIAN_POINT('Ctrl Pts',(-22.9314708233281,14.9100334467114,-8.77378154372893));
#37093=CARTESIAN_POINT('Ctrl Pts',(-22.92453848664,14.9615387374293,-8.63496920472942));
#37094=CARTESIAN_POINT('Ctrl Pts',(-22.917606149952,15.0069995860105,-8.49389673540899));
#37095=CARTESIAN_POINT('Ctrl Pts',(-22.9106738132639,15.0462379353463,-8.35110661131037));
#37096=CARTESIAN_POINT('Ctrl Pts',(-22.9037412290525,15.085477685711,-8.20831138880432));
#37097=CARTESIAN_POINT('Ctrl Pts',(-22.8968086448412,15.1184944014449,-8.06379870665251));
#37098=CARTESIAN_POINT('Ctrl Pts',(-22.8898760606299,15.1451601822359,-7.91812522911281));
#37099=CARTESIAN_POINT('Ctrl Pts',(-22.8829438499011,15.1718245264478,-7.77245959951431));
#37100=CARTESIAN_POINT('Ctrl Pts',(-22.8760116391724,15.1921385617596,-7.62563362499968));
#37101=CARTESIAN_POINT('Ctrl Pts',(-22.8690794284437,15.2060256970908,-7.47821318130803));
#37102=CARTESIAN_POINT('Ctrl Pts',(-22.8621456743553,15.2199159241982,-7.33075991651844));
#37103=CARTESIAN_POINT('Ctrl Pts',(-22.855211920267,15.2273763612686,-7.18271224732234));
#37104=CARTESIAN_POINT('Ctrl Pts',(-22.8482781661786,15.2283823298558,-7.03464081817565));
#37105=CARTESIAN_POINT('Ctrl Pts',(-22.8441608209693,15.2289796859043,-6.9467142517509));
#37106=CARTESIAN_POINT('Ctrl Pts',(-22.8400434757601,15.2273021079282,-6.85877936703632));
#37107=CARTESIAN_POINT('Ctrl Pts',(-22.8359261305508,15.223353127859,-6.77095565538246));
#37108=CARTESIAN_POINT('Ctrl Pts',(-22.8289927904143,15.2167033036104,-6.62306626695431));
#37109=CARTESIAN_POINT('Ctrl Pts',(-22.8220594502778,15.2036075003542,-6.47544108085083));
#37110=CARTESIAN_POINT('Ctrl Pts',(-22.8151261101414,15.1841106766401,-6.32864919185574));
#37111=CARTESIAN_POINT('Ctrl Pts',(-22.8081940903344,15.1646175657443,-6.18188525672731));
#37112=CARTESIAN_POINT('Ctrl Pts',(-22.8012620705275,15.1387259098974,-6.03595462967193));
#37113=CARTESIAN_POINT('Ctrl Pts',(-22.7943300507205,15.1065323796292,-5.8914199658471));
#37114=CARTESIAN_POINT('Ctrl Pts',(-22.7873977897876,15.0743377295293,-5.74688027447465));
#37115=CARTESIAN_POINT('Ctrl Pts',(-22.7804655288547,15.0358408349672,-5.60373696693589));
#37116=CARTESIAN_POINT('Ctrl Pts',(-22.7735332679218,14.9911893286948,-5.46254174975221));
#37117=CARTESIAN_POINT('Ctrl Pts',(-22.7666013833261,14.9465402464547,-5.32135419774698));
#37118=CARTESIAN_POINT('Ctrl Pts',(-22.7596694987304,14.8957373216521,-5.18211483944176));
#37119=CARTESIAN_POINT('Ctrl Pts',(-22.7527376141347,14.8389778369684,-5.04535949517476));
#37120=CARTESIAN_POINT('Ctrl Pts',(-22.7458041877542,14.7822057278808,-4.9085737338822));
#37121=CARTESIAN_POINT('Ctrl Pts',(-22.7388707613737,14.7194745384637,-4.77427339605927));
#37122=CARTESIAN_POINT('Ctrl Pts',(-22.7319373349933,14.6510296539597,-4.64297420710704));
#37123=CARTESIAN_POINT('Ctrl Pts',(-22.7278183852097,14.6103685108622,-4.56497312420261));
#37124=CARTESIAN_POINT('Ctrl Pts',(-22.7236994354262,14.5676917913382,-4.48803079706271));
#37125=CARTESIAN_POINT('Ctrl Pts',(-22.7195804856426,14.5230586438665,-4.4122512790253));
#37126=CARTESIAN_POINT('Ctrl Pts',(-22.7126467713343,14.4479245661251,-4.28468635201598));
#37127=CARTESIAN_POINT('Ctrl Pts',(-22.7057130570259,14.3672181299662,-4.16037389465996));
#37128=CARTESIAN_POINT('Ctrl Pts',(-22.6987793427176,14.2812456171528,-4.03979572825579));
#37129=CARTESIAN_POINT('Ctrl Pts',(-22.6960116860671,14.2469288878693,-3.99166583000592));
#37130=CARTESIAN_POINT('Ctrl Pts',(-22.6932440294166,14.2117736184024,-3.94413060177475));
#37131=CARTESIAN_POINT('Ctrl Pts',(-22.6904763727661,14.1758012177496,-3.89721939943571));
#37132=CARTESIAN_POINT('',(-23.534,5.20509380555675,-8.32288496556916));
#37133=CARTESIAN_POINT('Ctrl Pts',(-23.534,5.20509380555674,-8.3228849655691));
#37134=CARTESIAN_POINT('Ctrl Pts',(-23.4952181183639,5.41999536482199,-9.12285064450934));
#37135=CARTESIAN_POINT('Ctrl Pts',(-23.4176543550918,6.24677152044682,-10.6153578631701));
#37136=CARTESIAN_POINT('Ctrl Pts',(-23.3135388565479,8.1665770620453,-11.8658594947153));
#37137=CARTESIAN_POINT('Ctrl Pts',(-23.2482052396401,9.56246707210738,-12.0983697268913));
#37138=CARTESIAN_POINT('Ctrl Pts',(-23.2216535043684,10.1296134499674,-12.0988145792455));
#37139=CARTESIAN_POINT('',(-23.534,5.20511879703991,-5.67702200776683));
#37140=CARTESIAN_POINT('Origin',(-23.534,10.1295,-7.));
#37141=CARTESIAN_POINT('',(-23.0963464956316,10.1295667753203,-12.099051464939));
#37142=CARTESIAN_POINT('Ctrl Pts',(-23.534,5.20511879703991,-5.67702200776683));
#37143=CARTESIAN_POINT('Ctrl Pts',(-23.5270930683901,5.16684928138222,-5.81946858258322));
#37144=CARTESIAN_POINT('Ctrl Pts',(-23.5201861367802,5.13475838719278,-5.96360047114363));
#37145=CARTESIAN_POINT('Ctrl Pts',(-23.5132792051702,5.10897409853572,-6.10886551367019));
#37146=CARTESIAN_POINT('Ctrl Pts',(-23.5063724191029,5.08319035320424,-6.25412749517716));
#37147=CARTESIAN_POINT('Ctrl Pts',(-23.4994656330356,5.06371301191541,-6.40052225348957));
#37148=CARTESIAN_POINT('Ctrl Pts',(-23.4925588469683,5.05061883811789,-6.54748796316664));
#37149=CARTESIAN_POINT('Ctrl Pts',(-23.4856526672931,5.03752581394379,-6.69444076975995));
#37150=CARTESIAN_POINT('Ctrl Pts',(-23.4787464876178,5.03081486640317,-6.84196409317219));
#37151=CARTESIAN_POINT('Ctrl Pts',(-23.4718403079426,5.03051082838708,-6.98949153797166));
#37152=CARTESIAN_POINT('Ctrl Pts',(-23.4649324605092,5.03020671694952,-7.13705460884828));
#37153=CARTESIAN_POINT('Ctrl Pts',(-23.4580246130759,5.03631260848016,-7.28462146729374));
#37154=CARTESIAN_POINT('Ctrl Pts',(-23.4511167656425,5.04880119697882,-7.4316256166855));
#37155=CARTESIAN_POINT('Ctrl Pts',(-23.4457233772622,5.05855181882528,-7.54640094703876));
#37156=CARTESIAN_POINT('Ctrl Pts',(-23.4403299888818,5.07219222530019,-7.6608332110995));
#37157=CARTESIAN_POINT('Ctrl Pts',(-23.4349366005015,5.08968742686135,-7.77465490873909));
#37158=CARTESIAN_POINT('Ctrl Pts',(-23.4280029500233,5.11217896726539,-7.92098219181541));
#37159=CARTESIAN_POINT('Ctrl Pts',(-23.4210692995451,5.14105143184807,-8.06635446880544));
#37160=CARTESIAN_POINT('Ctrl Pts',(-23.4141356490668,5.17619897751155,-8.21021071744341));
#37161=CARTESIAN_POINT('Ctrl Pts',(-23.4072033126132,5.21133986221929,-8.35403970329283));
#37162=CARTESIAN_POINT('Ctrl Pts',(-23.4002709761595,5.25275337692516,-8.49635291307339));
#37163=CARTESIAN_POINT('Ctrl Pts',(-23.3933386397059,5.30028295761182,-8.63660128238601));
#37164=CARTESIAN_POINT('Ctrl Pts',(-23.3864060557303,5.34781423536222,-8.77685465932585));
#37165=CARTESIAN_POINT('Ctrl Pts',(-23.3794734717546,5.40146191313028,-8.9150427341364));
#37166=CARTESIAN_POINT('Ctrl Pts',(-23.372540887779,5.46101993551568,-9.05063280172548));
#37167=CARTESIAN_POINT('Ctrl Pts',(-23.3656086772861,5.5205747493001,-9.18621556459883));
#37168=CARTESIAN_POINT('Ctrl Pts',(-23.3586764667932,5.58603913675344,-9.31920029803885));
#37169=CARTESIAN_POINT('Ctrl Pts',(-23.3517442563004,5.65715938613674,-9.44907542423447));
#37170=CARTESIAN_POINT('Ctrl Pts',(-23.344810502446,5.72829546946732,-9.57897946534417));
#37171=CARTESIAN_POINT('Ctrl Pts',(-23.3378767485916,5.80508977194574,-9.70577222584034));
#37172=CARTESIAN_POINT('Ctrl Pts',(-23.3309429947373,5.8872429156988,-9.82896727282171));
#37173=CARTESIAN_POINT('Ctrl Pts',(-23.3268256483559,5.93602643992676,-9.90212197250362));
#37174=CARTESIAN_POINT('Ctrl Pts',(-23.3227083019746,5.98669870451527,-9.9740085792241));
#37175=CARTESIAN_POINT('Ctrl Pts',(-23.3185909555933,6.03918981564711,-10.0445301108347));
#37176=CARTESIAN_POINT('Ctrl Pts',(-23.3116576154912,6.12758138927418,-10.1632837249084));
#37177=CARTESIAN_POINT('Ctrl Pts',(-23.3047242753892,6.2211633857878,-10.2782058956995));
#37178=CARTESIAN_POINT('Ctrl Pts',(-23.2977909352871,6.31957962315759,-10.3888505015891));
#37179=CARTESIAN_POINT('Ctrl Pts',(-23.2908589155155,6.41797711891773,-10.4994740371954));
#37180=CARTESIAN_POINT('Ctrl Pts',(-23.2839268957439,6.52120679919802,-10.6058213862124));
#37181=CARTESIAN_POINT('Ctrl Pts',(-23.2769948759722,6.62887326370307,-10.7074807421109));
#37182=CARTESIAN_POINT('Ctrl Pts',(-23.2700626150757,6.73654347330243,-10.8091436341511));
#37183=CARTESIAN_POINT('Ctrl Pts',(-23.2631303541791,6.84865053786333,-10.9061179773462));
#37184=CARTESIAN_POINT('Ctrl Pts',(-23.2561980932826,6.96476298683145,-10.9980295943728));
#37185=CARTESIAN_POINT('Ctrl Pts',(-23.2492662087238,7.08086913230112,-11.0899362217128));
#37186=CARTESIAN_POINT('Ctrl Pts',(-23.242334324165,7.20097996725761,-11.1767804683628));
#37187=CARTESIAN_POINT('Ctrl Pts',(-23.2354024396061,7.32463180495147,-11.2582291399601));
#37188=CARTESIAN_POINT('Ctrl Pts',(-23.228469013263,7.44831114519037,-11.3396959273073));
#37189=CARTESIAN_POINT('Ctrl Pts',(-23.2215355869198,7.57553278566364,-11.4157645597463));
#37190=CARTESIAN_POINT('Ctrl Pts',(-23.2146021605767,7.70580446372751,-11.4861454443044));
#37191=CARTESIAN_POINT('Ctrl Pts',(-23.2104832106128,7.78319513568321,-11.5279567115709));
#37192=CARTESIAN_POINT('Ctrl Pts',(-23.206364260649,7.86166171055427,-11.5677615028387));
#37193=CARTESIAN_POINT('Ctrl Pts',(-23.2022453106851,7.94109688570871,-11.6055067918048));
#37194=CARTESIAN_POINT('Ctrl Pts',(-23.1953326013538,8.0744105412136,-11.6688535703621));
#37195=CARTESIAN_POINT('Ctrl Pts',(-23.1884198920225,8.21050236448007,-11.7264202219746));
#37196=CARTESIAN_POINT('Ctrl Pts',(-23.1815071826912,8.34885199561309,-11.7779800841436));
#37197=CARTESIAN_POINT('Ctrl Pts',(-23.1744104587696,8.49088445926188,-11.8309124569247));
#37198=CARTESIAN_POINT('Ctrl Pts',(-23.1673137348479,8.63529628394864,-11.8775136191942));
#37199=CARTESIAN_POINT('Ctrl Pts',(-23.1602170109263,8.78150369622116,-11.9175915817602));
#37200=CARTESIAN_POINT('Ctrl Pts',(-23.1533056463726,8.92389231635461,-11.9566227478196));
#37201=CARTESIAN_POINT('Ctrl Pts',(-23.1463942818189,9.06798355227891,-11.9894671549689));
#37202=CARTESIAN_POINT('Ctrl Pts',(-23.1394829172652,9.21322389390579,-12.0159983151314));
#37203=CARTESIAN_POINT('Ctrl Pts',(-23.1322935136596,9.36430714637444,-12.0435968041202));
#37204=CARTESIAN_POINT('Ctrl Pts',(-23.125104110054,9.51663350849815,-12.0643634281151));
#37205=CARTESIAN_POINT('Ctrl Pts',(-23.1179147064484,9.66956947446774,-12.0782147366652));
#37206=CARTESIAN_POINT('Ctrl Pts',(-23.1107253028428,9.82250544043734,-12.0920660452153));
#37207=CARTESIAN_POINT('Ctrl Pts',(-23.1035358992372,9.97605060390634,-12.0990020099546));
#37208=CARTESIAN_POINT('Ctrl Pts',(-23.0963464956316,10.1295667746463,-12.0989999995628));
#37209=CARTESIAN_POINT('Ctrl Pts',(-23.0963464956316,10.129566778808,-12.099317792417));
#37210=CARTESIAN_POINT('Ctrl Pts',(-23.0928642190133,10.2039288711016,-12.0993673408814));
#37211=CARTESIAN_POINT('Ctrl Pts',(-23.0506000607591,11.1064308613037,-12.0800148219986));
#37212=CARTESIAN_POINT('Ctrl Pts',(-22.9695540208687,12.8165649252773,-11.5744658007328));
#37213=CARTESIAN_POINT('Ctrl Pts',(-22.8532083759605,14.6458800384554,-9.78358876962574));
#37214=CARTESIAN_POINT('Ctrl Pts',(-22.7368627310523,15.4235830862095,-7.34457044966851));
#37215=CARTESIAN_POINT('Ctrl Pts',(-22.640850630295,15.0481127832734,-5.26560594787934));
#37216=CARTESIAN_POINT('Ctrl Pts',(-22.5836204111736,14.4153514965049,-4.21017316538278));
#37217=CARTESIAN_POINT('Ctrl Pts',(-22.5651720736884,14.1754919335065,-3.89745664672419));
#37218=CARTESIAN_POINT('Origin',(26.8463464956315,10.1295,-7.));
#37219=CARTESIAN_POINT('',(18.1904820160362,6.08319878352125,-3.8972193977784));
#37220=CARTESIAN_POINT('',(18.0651682149652,6.08305061783963,-3.89710564634619));
#37221=CARTESIAN_POINT('',(26.8463464956315,6.08319878352126,-3.89721939777839));
#37222=CARTESIAN_POINT('',(17.734,12.4414757859806,-2.45527019889635));
#37223=CARTESIAN_POINT('Ctrl Pts',(18.0651682149652,6.08305061783963,-3.89710564634619));
#37224=CARTESIAN_POINT('Ctrl Pts',(18.0323425732489,6.51012300040625,-3.34120496454716));
#37225=CARTESIAN_POINT('Ctrl Pts',(17.9607350498965,7.69350565290941,-2.32091790294544));
#37226=CARTESIAN_POINT('Ctrl Pts',(17.8503456449082,10.0408176861101,-1.69542432103654));
#37227=CARTESIAN_POINT('Ctrl Pts',(17.772781881636,11.703188220458,-2.0796916608358));
#37228=CARTESIAN_POINT('Ctrl Pts',(17.734,12.4414757859806,-2.45527019889635));
#37229=CARTESIAN_POINT('',(17.734,14.4077184404108,-4.2257166734219));
#37230=CARTESIAN_POINT('Origin',(17.734,10.1295,-7.));
#37231=CARTESIAN_POINT('Ctrl Pts',(18.1904820160362,6.08319878352125,-3.89721939777841));
#37232=CARTESIAN_POINT('Ctrl Pts',(18.1876881220985,6.11950371475326,-3.84987454609825));
#37233=CARTESIAN_POINT('Ctrl Pts',(18.1848942281607,6.15663752372707,-3.80316978774102));
#37234=CARTESIAN_POINT('Ctrl Pts',(18.182100334223,6.19457664874617,-3.75713410395105));
#37235=CARTESIAN_POINT('Ctrl Pts',(18.1751666155273,6.28873169768777,-3.6428855002175));
#37236=CARTESIAN_POINT('Ctrl Pts',(18.1682328968315,6.38788205597123,-3.53272058770171));
#37237=CARTESIAN_POINT('Ctrl Pts',(18.1612991781358,6.49164988118888,-3.42706737915953));
#37238=CARTESIAN_POINT('Ctrl Pts',(18.1543667758962,6.59539800474323,-3.32143423024506));
#37239=CARTESIAN_POINT('Ctrl Pts',(18.1474343736566,6.70376161461654,-3.22031131194671));
#37240=CARTESIAN_POINT('Ctrl Pts',(18.140501971417,6.81632539466393,-3.12409042487364));
#37241=CARTESIAN_POINT('Ctrl Pts',(18.133569325952,6.92889312404448,-3.0278661618626));
#37242=CARTESIAN_POINT('Ctrl Pts',(18.1266366804871,7.0456610693994,-2.93654449155152));
#37243=CARTESIAN_POINT('Ctrl Pts',(18.1197040350221,7.16617974834539,-2.85047784845849));
#37244=CARTESIAN_POINT('Ctrl Pts',(18.1127717656245,7.28669188965202,-2.76441587412453));
#37245=CARTESIAN_POINT('Ctrl Pts',(18.1058394962268,7.41095408788024,-2.6836085479493));
#37246=CARTESIAN_POINT('Ctrl Pts',(18.0989072268292,7.538486708999,-2.60836577959227));
#37247=CARTESIAN_POINT('Ctrl Pts',(18.0919734185825,7.66604764024758,-2.53310630858678));
#37248=CARTESIAN_POINT('Ctrl Pts',(18.0850396103359,7.796880160196,-2.46341403160095));
#37249=CARTESIAN_POINT('Ctrl Pts',(18.0781058020892,7.93047824811605,-2.39955389828973));
#37250=CARTESIAN_POINT('Ctrl Pts',(18.0739887644978,8.00980382657902,-2.36163612495553));
#37251=CARTESIAN_POINT('Ctrl Pts',(18.0698717269063,8.09010394201909,-2.3257736263611));
#37252=CARTESIAN_POINT('Ctrl Pts',(18.0657546893148,8.17126896360323,-2.29201399661252));
#37253=CARTESIAN_POINT('Ctrl Pts',(18.0588213573683,8.30795560407876,-2.2351608068521));
#37254=CARTESIAN_POINT('Ctrl Pts',(18.0518880254217,8.44714343822144,-2.18425443098161));
#37255=CARTESIAN_POINT('Ctrl Pts',(18.0449546934752,8.58829824151367,-2.13949610229159));
#37256=CARTESIAN_POINT('Ctrl Pts',(18.0380226783627,8.72942623555296,-2.09474627446251));
#37257=CARTESIAN_POINT('Ctrl Pts',(18.0310906632502,8.87252013840123,-2.0561422639854));
#37258=CARTESIAN_POINT('Ctrl Pts',(18.0241586481377,9.01702957132649,-2.02383575981188));
#37259=CARTESIAN_POINT('Ctrl Pts',(18.0172263866156,9.16154414107234,-1.99152810725164));
#37260=CARTESIAN_POINT('Ctrl Pts',(18.0102941250934,9.30747401965934,-1.96551848432784));
#37261=CARTESIAN_POINT('Ctrl Pts',(18.0033618635713,9.45425707373931,-1.94590779758275));
#37262=CARTESIAN_POINT('Ctrl Pts',(17.9964299753957,9.60103222261469,-1.92629816699833));
#37263=CARTESIAN_POINT('Ctrl Pts',(17.9894980872201,9.74866012719367,-1.9130868258486));
#37264=CARTESIAN_POINT('Ctrl Pts',(17.9825661990445,9.89657192712221,-1.9063229869901));
#37265=CARTESIAN_POINT('Ctrl Pts',(17.9756327645019,10.0445167232454,-1.89955763925304));
#37266=CARTESIAN_POINT('Ctrl Pts',(17.9686993299592,10.1927452108641,-1.89924268284508));
#37267=CARTESIAN_POINT('Ctrl Pts',(17.9617658954166,10.3406862695542,-1.90537524840624));
#37268=CARTESIAN_POINT('Ctrl Pts',(17.9576469450799,10.4285737183722,-1.90901842594365));
#37269=CARTESIAN_POINT('Ctrl Pts',(17.9535279947433,10.5163597158814,-1.9149360686311));
#37270=CARTESIAN_POINT('Ctrl Pts',(17.9494090444066,10.6039249349976,-1.92311887266872));
#37271=CARTESIAN_POINT('Ctrl Pts',(17.9424753834828,10.7513283966681,-1.93689344724857));
#37272=CARTESIAN_POINT('Ctrl Pts',(17.9355417225589,10.8981569837258,-1.9570943475134));
#37273=CARTESIAN_POINT('Ctrl Pts',(17.9286080616351,11.043844383057,-1.98364919994901));
#37274=CARTESIAN_POINT('Ctrl Pts',(17.921675718497,11.1895040935834,-2.01019900546824));
#37275=CARTESIAN_POINT('Ctrl Pts',(17.914743375359,11.3340227240848,-2.04310029455465));
#37276=CARTESIAN_POINT('Ctrl Pts',(17.9078110322209,11.4768428889456,-2.08222935268351));
#37277=CARTESIAN_POINT('Ctrl Pts',(17.9008784472619,11.6196680358023,-2.12135977575131));
#37278=CARTESIAN_POINT('Ctrl Pts',(17.893945862303,11.760794278772,-2.16671831846166));
#37279=CARTESIAN_POINT('Ctrl Pts',(17.887013277344,11.8996776268284,-2.2181308916412));
#37280=CARTESIAN_POINT('Ctrl Pts',(17.8800810690987,12.0385534280233,-2.26954067108361));
#37281=CARTESIAN_POINT('Ctrl Pts',(17.8731488608534,12.1751862684927,-2.32700370709501));
#37282=CARTESIAN_POINT('Ctrl Pts',(17.8662166526081,12.3090504196554,-2.3902970846073));
#37283=CARTESIAN_POINT('Ctrl Pts',(17.8592829059654,12.4429442779832,-2.45360450820139));
#37284=CARTESIAN_POINT('Ctrl Pts',(17.8523491593228,12.5740679203451,-2.52274471727729));
#37285=CARTESIAN_POINT('Ctrl Pts',(17.8454154126802,12.7019180096239,-2.59744771936065));
#37286=CARTESIAN_POINT('Ctrl Pts',(17.8412980749529,12.7778368487668,-2.64180721281625));
#37287=CARTESIAN_POINT('Ctrl Pts',(17.8371807372257,12.8526018488398,-2.68812732988671));
#37288=CARTESIAN_POINT('Ctrl Pts',(17.8330633994984,12.9261120521225,-2.73634405352367));
#37289=CARTESIAN_POINT('Ctrl Pts',(17.8261558289376,13.0494385678835,-2.8172362325956));
#37290=CARTESIAN_POINT('Ctrl Pts',(17.8192482583768,13.1692774271192,-2.90349891677528));
#37291=CARTESIAN_POINT('Ctrl Pts',(17.812340687816,13.2851650747901,-2.99480600522892));
#37292=CARTESIAN_POINT('Ctrl Pts',(17.805433747039,13.4010421566397,-3.08610476894398));
#37293=CARTESIAN_POINT('Ctrl Pts',(17.7985268062619,13.512968479376,-3.18244681517665));
#37294=CARTESIAN_POINT('Ctrl Pts',(17.7916198654848,13.6205122246208,-3.28346469846606));
#37295=CARTESIAN_POINT('Ctrl Pts',(17.7847138003811,13.728042335292,-3.38446977454133));
#37296=CARTESIAN_POINT('Ctrl Pts',(17.7778077352774,13.8311907337587,-3.49014927375184));
#37297=CARTESIAN_POINT('Ctrl Pts',(17.7709016701737,13.929561225329,-3.60009769496956));
#37298=CARTESIAN_POINT('Ctrl Pts',(17.7639943665765,14.0279493580916,-3.71006583369829));
#37299=CARTESIAN_POINT('Ctrl Pts',(17.7570870629792,14.1215576465777,-3.82430417516951));
#37300=CARTESIAN_POINT('Ctrl Pts',(17.7501797593819,14.2100286837041,-3.94237238018294));
#37301=CARTESIAN_POINT('Ctrl Pts',(17.7447865062546,14.2791072598717,-4.03456055563452));
#37302=CARTESIAN_POINT('Ctrl Pts',(17.7393932531273,14.3450546292517,-4.12908289781627));
#37303=CARTESIAN_POINT('Ctrl Pts',(17.734,14.4077184404108,-4.2257166734219));
#37304=CARTESIAN_POINT('Origin',(26.8463464956315,10.1295,-7.));
#37305=CARTESIAN_POINT('',(19.690497962139,6.0828868892326,-3.89698012451499));
#37306=CARTESIAN_POINT('',(19.5651698457322,6.08319878352126,-3.8972193977784));
#37307=CARTESIAN_POINT('',(26.8463464956315,6.08319878352126,-3.89721939777839));
#37308=CARTESIAN_POINT('',(18.5963464953293,10.1294414208446,-12.0989827726088));
#37309=CARTESIAN_POINT('Ctrl Pts',(19.5651698457322,6.08319878352126,-3.8972193977784));
#37310=CARTESIAN_POINT('Ctrl Pts',(19.5580044147231,6.17633171704041,-3.77576578874045));
#37311=CARTESIAN_POINT('Ctrl Pts',(19.550838983714,6.2749444499284,-3.65849855722346));
#37312=CARTESIAN_POINT('Ctrl Pts',(19.5436735527049,6.37863283527319,-3.54590149060942));
#37313=CARTESIAN_POINT('Ctrl Pts',(19.5367389813393,6.47898053341559,-3.43693213579948));
#37314=CARTESIAN_POINT('Ctrl Pts',(19.5298044099736,6.58408164185059,-3.3323369197218));
#37315=CARTESIAN_POINT('Ctrl Pts',(19.522869838608,6.69353073715527,-3.23251858335224));
#37316=CARTESIAN_POINT('Ctrl Pts',(19.5155889777771,6.80844535681325,-3.12771565074809));
#37317=CARTESIAN_POINT('Ctrl Pts',(19.5083081169463,6.92815308930806,-3.02817921830671));
#37318=CARTESIAN_POINT('Ctrl Pts',(19.5010272561154,7.05214335024002,-2.93432944642854));
#37319=CARTESIAN_POINT('Ctrl Pts',(19.4937463952846,7.17613361117198,-2.84047967455038));
#37320=CARTESIAN_POINT('Ctrl Pts',(19.4864655344537,7.3044060595409,-2.75231680996947));
#37321=CARTESIAN_POINT('Ctrl Pts',(19.4791846736229,7.43641261061583,-2.67021001512314));
#37322=CARTESIAN_POINT('Ctrl Pts',(19.4722525172567,7.56209693210968,-2.59203558577654));
#37323=CARTESIAN_POINT('Ctrl Pts',(19.4653203608905,7.69120946211311,-2.51932363092219));
#37324=CARTESIAN_POINT('Ctrl Pts',(19.4583882045243,7.82325572183359,-2.45235903688245));
#37325=CARTESIAN_POINT('Ctrl Pts',(19.4514573849167,7.95527651848407,-2.38540735592446));
#37326=CARTESIAN_POINT('Ctrl Pts',(19.4445265653092,8.09022962124302,-2.32420097417425));
#37327=CARTESIAN_POINT('Ctrl Pts',(19.4375957457017,8.22759659625989,-2.26897849900872));
#37328=CARTESIAN_POINT('Ctrl Pts',(19.4306646979627,8.36496809278,-2.21375420616758));
#37329=CARTESIAN_POINT('Ctrl Pts',(19.4237336502237,8.50475331485513,-2.1645143406319));
#37330=CARTESIAN_POINT('Ctrl Pts',(19.4168026024848,8.64641401791106,-2.12144929618116));
#37331=CARTESIAN_POINT('Ctrl Pts',(19.4098719355473,8.78806693792943,-2.07838661778433));
#37332=CARTESIAN_POINT('Ctrl Pts',(19.4029412686098,8.93159481592084,-2.04149817701049));
#37333=CARTESIAN_POINT('Ctrl Pts',(19.3960106016723,9.07644441149005,-2.01092444159161));
#37334=CARTESIAN_POINT('Ctrl Pts',(19.3890783892253,9.22132630791031,-1.98034388835823));
#37335=CARTESIAN_POINT('Ctrl Pts',(19.3821461767782,9.36753018698962,-1.95608092251631));
#37336=CARTESIAN_POINT('Ctrl Pts',(19.3752139643311,9.51449215978502,-1.93822497966631));
#37337=CARTESIAN_POINT('Ctrl Pts',(19.3710889857923,9.60194115077149,-1.92759988968118));
#37338=CARTESIAN_POINT('Ctrl Pts',(19.3669640072535,9.68965839362785,-1.91924240856535));
#37339=CARTESIAN_POINT('Ctrl Pts',(19.3628390287147,9.77752407795016,-1.91316267703624));
#37340=CARTESIAN_POINT('Ctrl Pts',(19.3559048075467,9.9252291102158,-1.90294245342334));
#37341=CARTESIAN_POINT('Ctrl Pts',(19.3489705863787,10.0734048576221,-1.89915811700655));
#37342=CARTESIAN_POINT('Ctrl Pts',(19.3420363652107,10.2214806592299,-1.9018296852373));
#37343=CARTESIAN_POINT('Ctrl Pts',(19.335103451794,10.3695285346548,-1.90450074962676));
#37344=CARTESIAN_POINT('Ctrl Pts',(19.3281705383774,10.5174761716726,-1.91362528350658));
#37345=CARTESIAN_POINT('Ctrl Pts',(19.3212376249607,10.6647534305791,-1.92917119545007));
#37346=CARTESIAN_POINT('Ctrl Pts',(19.3143044602487,10.8120360278019,-1.94471767088173));
#37347=CARTESIAN_POINT('Ctrl Pts',(19.3073712955368,10.9586478693285,-1.96668595872507));
#37348=CARTESIAN_POINT('Ctrl Pts',(19.3004381308248,11.1040238996176,-1.99499209100783));
#37349=CARTESIAN_POINT('Ctrl Pts',(19.2935053388582,11.2493921141048,-2.02329670147767));
#37350=CARTESIAN_POINT('Ctrl Pts',(19.2865725468916,11.3935243261183,-2.05793841047807));
#37351=CARTESIAN_POINT('Ctrl Pts',(19.279639754925,11.535865618028,-2.09878211579726));
#37352=CARTESIAN_POINT('Ctrl Pts',(19.2727054235545,11.678238516357,-2.13963489032792));
#37353=CARTESIAN_POINT('Ctrl Pts',(19.2657710921841,11.8188193822447,-2.18669232169525));
#37354=CARTESIAN_POINT('Ctrl Pts',(19.2588367608137,11.9570677921862,-2.23976923196325));
#37355=CARTESIAN_POINT('Ctrl Pts',(19.2547223018113,12.0390969575754,-2.27126221370942));
#37356=CARTESIAN_POINT('Ctrl Pts',(19.2506078428089,12.1203052653314,-2.30487346637448));
#37357=CARTESIAN_POINT('Ctrl Pts',(19.2464933838065,12.2005829824517,-2.34055622635073));
#37358=CARTESIAN_POINT('Ctrl Pts',(19.2395600659607,12.3358598021767,-2.40068561793972));
#37359=CARTESIAN_POINT('Ctrl Pts',(19.2326267481149,12.4685396684855,-2.4667205822027));
#37360=CARTESIAN_POINT('Ctrl Pts',(19.225693430269,12.5981090877672,-2.53841169853235));
#37361=CARTESIAN_POINT('Ctrl Pts',(19.2187614321196,12.7276538446444,-2.6100891690857));
#37362=CARTESIAN_POINT('Ctrl Pts',(19.2118294339701,12.8540890465733,-2.68742048375259));
#37363=CARTESIAN_POINT('Ctrl Pts',(19.2048974358206,12.9769260564387,-2.77011042069487));
#37364=CARTESIAN_POINT('Ctrl Pts',(19.1979651953757,13.0997673598497,-2.85280324791448));
#37365=CARTESIAN_POINT('Ctrl Pts',(19.1910329549307,13.2190099433899,-2.9408548903621));
#37366=CARTESIAN_POINT('Ctrl Pts',(19.1841007144858,13.3341939513471,-3.03392666757164));
#37367=CARTESIAN_POINT('Ctrl Pts',(19.1771688496638,13.4493717180665,-3.12699340169313));
#37368=CARTESIAN_POINT('Ctrl Pts',(19.1702369848419,13.5604910926603,-3.22507951774791));
#37369=CARTESIAN_POINT('Ctrl Pts',(19.1633051200199,13.667125119773,-3.3278058994722));
#37370=CARTESIAN_POINT('Ctrl Pts',(19.1563717121302,13.7737828841536,-3.430555148603));
#37371=CARTESIAN_POINT('Ctrl Pts',(19.1494383042404,13.8759530677986,-3.53794649789823));
#37372=CARTESIAN_POINT('Ctrl Pts',(19.1425048963507,13.9732449701325,-3.64956337105432));
#37373=CARTESIAN_POINT('Ctrl Pts',(19.1383858438666,14.0310448945516,-3.71587358472634));
#37374=CARTESIAN_POINT('Ctrl Pts',(19.1342667913824,14.0871237909435,-3.78367446321953));
#37375=CARTESIAN_POINT('Ctrl Pts',(19.1301477388983,14.1414063406675,-3.85287297464629));
#37376=CARTESIAN_POINT('Ctrl Pts',(19.1232141285398,14.2327802793352,-3.96935498536888));
#37377=CARTESIAN_POINT('Ctrl Pts',(19.1162805181812,14.3190936323279,-4.08983919704816));
#37378=CARTESIAN_POINT('Ctrl Pts',(19.1093469078227,14.400009475508,-4.213864716207));
#37379=CARTESIAN_POINT('Ctrl Pts',(19.1024146136957,14.4809099581506,-4.3378666911678));
#37380=CARTESIAN_POINT('Ctrl Pts',(19.0954823195687,14.5564147947404,-4.46540835564231));
#37381=CARTESIAN_POINT('Ctrl Pts',(19.0885500254416,14.6262304728754,-4.59599998870346));
#37382=CARTESIAN_POINT('Ctrl Pts',(19.0816174867073,14.6960486144694,-4.72659622971433));
#37383=CARTESIAN_POINT('Ctrl Pts',(19.0746849479731,14.7601770371195,-4.86024236471895));
#37384=CARTESIAN_POINT('Ctrl Pts',(19.0677524092388,14.8183680106684,-4.99642375275354));
#37385=CARTESIAN_POINT('Ctrl Pts',(19.0608202455346,14.8765558362549,-5.13259777377116));
#37386=CARTESIAN_POINT('Ctrl Pts',(19.0538880818305,14.928806726421,-5.2713064690269));
#37387=CARTESIAN_POINT('Ctrl Pts',(19.0469559181264,14.9749209568293,-5.41201487692134));
#37388=CARTESIAN_POINT('Ctrl Pts',(19.0400222130546,15.0210454407442,-5.55275457135289));
#37389=CARTESIAN_POINT('Ctrl Pts',(19.0330885079828,15.061030435488,-5.69549455262194));
#37390=CARTESIAN_POINT('Ctrl Pts',(19.0261548029109,15.0947257927471,-5.83968373835435));
#37391=CARTESIAN_POINT('Ctrl Pts',(19.0220372332707,15.1147357266325,-5.92531025512671));
#37392=CARTESIAN_POINT('Ctrl Pts',(19.0179196636304,15.1325285371395,-6.01144756489171));
#37393=CARTESIAN_POINT('Ctrl Pts',(19.0138020939901,15.1480812641024,-6.09797832864145));
#37394=CARTESIAN_POINT('Ctrl Pts',(19.0068685366312,15.1742704324482,-6.243687100122));
#37395=CARTESIAN_POINT('Ctrl Pts',(18.9999349792723,15.1941141114036,-6.39056233036988));
#37396=CARTESIAN_POINT('Ctrl Pts',(18.9930014219134,15.2075304301788,-6.53803901660621));
#37397=CARTESIAN_POINT('Ctrl Pts',(18.9860691810523,15.2209442015525,-6.68548770094879));
#37398=CARTESIAN_POINT('Ctrl Pts',(18.9791369401912,15.2279330176624,-6.83353728439083));
#37399=CARTESIAN_POINT('Ctrl Pts',(18.9722046993301,15.2284668647841,-6.98161762166019));
#37400=CARTESIAN_POINT('Ctrl Pts',(18.9652722137388,15.2290007307523,-7.12970318663658));
#37401=CARTESIAN_POINT('Ctrl Pts',(18.9583397281476,15.2230791672004,-7.27781917705496));
#37402=CARTESIAN_POINT('Ctrl Pts',(18.9514072425563,15.2107242822434,-7.42539486778765));
#37403=CARTESIAN_POINT('Ctrl Pts',(18.944475131797,15.1983700653015,-7.57296257926424));
#37404=CARTESIAN_POINT('Ctrl Pts',(18.9375430210376,15.1795832514988,-7.71998972015298));
#37405=CARTESIAN_POINT('Ctrl Pts',(18.9306109102783,15.1544378816705,-7.86591009080227));
#37406=CARTESIAN_POINT('Ctrl Pts',(18.9236772573793,15.1292869179224,-8.01186292336624));
#37407=CARTESIAN_POINT('Ctrl Pts',(18.9167436044803,15.0977746278606,-8.1567081678229));
#37408=CARTESIAN_POINT('Ctrl Pts',(18.9098099515813,15.0600264057109,-8.29988859622186));
#37409=CARTESIAN_POINT('Ctrl Pts',(18.9056921174149,15.0376080756969,-8.38492216635026));
#37410=CARTESIAN_POINT('Ctrl Pts',(18.9015742832484,15.0129912650688,-8.46936874673093));
#37411=CARTESIAN_POINT('Ctrl Pts',(18.8974564490819,14.9862106421525,-8.55311388455654));
#37412=CARTESIAN_POINT('Ctrl Pts',(18.8905228749338,14.94111765705,-8.69412323539135));
#37413=CARTESIAN_POINT('Ctrl Pts',(18.8835893007856,14.8898716746156,-8.83319174903818));
#37414=CARTESIAN_POINT('Ctrl Pts',(18.8766557266375,14.832664936967,-8.96978185992368));
#37415=CARTESIAN_POINT('Ctrl Pts',(18.8697234694038,14.7754690647647,-9.10634602784188));
#37416=CARTESIAN_POINT('Ctrl Pts',(18.8627912121701,14.7123148237805,-9.2404324274278));
#37417=CARTESIAN_POINT('Ctrl Pts',(18.8558589549363,14.6434426840965,-9.37152323300689));
#37418=CARTESIAN_POINT('Ctrl Pts',(18.8489264537584,14.5745681208209,-9.50261865163537));
#37419=CARTESIAN_POINT('Ctrl Pts',(18.8419939525805,14.4999754069997,-9.6307179711243));
#37420=CARTESIAN_POINT('Ctrl Pts',(18.8350614514025,14.419951338008,-9.75532726117709));
#37421=CARTESIAN_POINT('Ctrl Pts',(18.8281293255397,14.3399316013977,-9.87992980507238));
#37422=CARTESIAN_POINT('Ctrl Pts',(18.8211971996768,14.254481277422,-10.0010424199487));
#37423=CARTESIAN_POINT('Ctrl Pts',(18.8142650738139,14.1639309289768,-10.1181994931876));
#37424=CARTESIAN_POINT('Ctrl Pts',(18.8073314066908,14.0733604479404,-10.2353826146473));
#37425=CARTESIAN_POINT('Ctrl Pts',(18.8003977395676,13.9776878789461,-10.3486081755401));
#37426=CARTESIAN_POINT('Ctrl Pts',(18.7934640724445,13.8772849584178,-10.4574425382726));
#37427=CARTESIAN_POINT('Ctrl Pts',(18.7893463163542,13.8176578188189,-10.5220769304364));
#37428=CARTESIAN_POINT('Ctrl Pts',(18.785228560264,13.7563630890054,-10.5851632174693));
#37429=CARTESIAN_POINT('Ctrl Pts',(18.7811108041737,13.6934849922401,-10.6466165105598));
#37430=CARTESIAN_POINT('Ctrl Pts',(18.7741773221436,13.5876107868588,-10.7500916300169));
#37431=CARTESIAN_POINT('Ctrl Pts',(18.7672438401135,13.4772089013387,-10.8489706438041));
#37432=CARTESIAN_POINT('Ctrl Pts',(18.7603103580834,13.3627009182633,-10.9428686032052));
#37433=CARTESIAN_POINT('Ctrl Pts',(18.7533781928252,13.2482146819653,-11.0367487299805));
#37434=CARTESIAN_POINT('Ctrl Pts',(18.7464460275669,13.1296241594458,-11.125649480223));
#37435=CARTESIAN_POINT('Ctrl Pts',(18.7395138623087,13.0073843026664,-11.2092259312689));
#37436=CARTESIAN_POINT('Ctrl Pts',(18.7325814519985,12.8851401247102,-11.2928053367408));
#37437=CARTESIAN_POINT('Ctrl Pts',(18.7256490416884,12.7592466253657,-11.3710598770506));
#37438=CARTESIAN_POINT('Ctrl Pts',(18.7187166313782,12.6301884988541,-11.443687436319));
#37439=CARTESIAN_POINT('Ctrl Pts',(18.7117845955379,12.5011373437089,-11.5163110724455));
#37440=CARTESIAN_POINT('Ctrl Pts',(18.7048525596975,12.3689221920308,-11.5833081744225));
#37441=CARTESIAN_POINT('Ctrl Pts',(18.6979205238572,12.2340531491347,-11.6444221430084));
#37442=CARTESIAN_POINT('Ctrl Pts',(18.6909869446661,12.0991540789498,-11.7055497180288));
#37443=CARTESIAN_POINT('Ctrl Pts',(18.684053365475,11.9616002381559,-11.7607914059617));
#37444=CARTESIAN_POINT('Ctrl Pts',(18.6771197862838,11.8219231385118,-11.8099381409983));
#37445=CARTESIAN_POINT('Ctrl Pts',(18.6730015772777,11.7389617308688,-11.8391289126429));
#37446=CARTESIAN_POINT('Ctrl Pts',(18.6688833682717,11.6552516632413,-11.8661704363263));
#37447=CARTESIAN_POINT('Ctrl Pts',(18.6647651592656,11.5709071450112,-11.891027135716));
#37448=CARTESIAN_POINT('Ctrl Pts',(18.6577998246933,11.4282510078553,-11.9330685249111));
#37449=CARTESIAN_POINT('Ctrl Pts',(18.650834490121,11.2837317271447,-11.9688711473952));
#37450=CARTESIAN_POINT('Ctrl Pts',(18.6438691555487,11.1379071299167,-11.9982913140726));
#37451=CARTESIAN_POINT('Ctrl Pts',(18.6369053523104,10.9921145923347,-12.0277050127044));
#37452=CARTESIAN_POINT('Ctrl Pts',(18.6299415490721,10.8450176285976,-12.0507389918283));
#37453=CARTESIAN_POINT('Ctrl Pts',(18.6229777458338,10.6971847677683,-12.0673005638549));
#37454=CARTESIAN_POINT('Ctrl Pts',(18.6160146892149,10.5493677567394,-12.0838603602436));
#37455=CARTESIAN_POINT('Ctrl Pts',(18.609051632596,10.4008153280418,-12.0939490974492));
#37456=CARTESIAN_POINT('Ctrl Pts',(18.6020885759772,10.2521021089812,-12.0975258432767));
#37457=CARTESIAN_POINT('Ctrl Pts',(18.6001745491953,10.2112233541923,-12.0985090303568));
#37458=CARTESIAN_POINT('Ctrl Pts',(18.5982605224134,10.1703324708191,-12.0990004693845));
#37459=CARTESIAN_POINT('Ctrl Pts',(18.5963464956315,10.1294414271024,-12.0989999996636));
#37460=CARTESIAN_POINT('Ctrl Pts',(18.5963464895963,10.1294413021288,-12.0986559623714));
#37461=CARTESIAN_POINT('Ctrl Pts',(18.5803708311834,9.78816223566316,-12.0988021887428));
#37462=CARTESIAN_POINT('Ctrl Pts',(18.5256132911343,8.61850505157706,-11.9829820583334));
#37463=CARTESIAN_POINT('Ctrl Pts',(18.4320738694491,6.76024937160752,-11.0980785162391));
#37464=CARTESIAN_POINT('Ctrl Pts',(18.3157282245409,5.23345505271711,-9.04320502425034));
#37465=CARTESIAN_POINT('Ctrl Pts',(18.1993825796327,4.8466304876897,-6.51259606632921));
#37466=CARTESIAN_POINT('Ctrl Pts',(18.1158625764408,5.45203935924674,-4.777421692593));
#37467=CARTESIAN_POINT('Ctrl Pts',(18.071124454885,6.00555797974676,-3.99797428620377));
#37468=CARTESIAN_POINT('Ctrl Pts',(18.0651682149652,6.08305061783963,-3.89710564634619));
#37469=CARTESIAN_POINT('',(18.721653505176,10.1295871904926,-12.0989689030608));
#37470=CARTESIAN_POINT('Ctrl Pts',(18.7216535043684,10.1295871737727,-12.0989999992548));
#37471=CARTESIAN_POINT('Ctrl Pts',(18.7147113410273,9.98128307520553,-12.0990025346986));
#37472=CARTESIAN_POINT('Ctrl Pts',(18.7077691776862,9.8329749558716,-12.0925306029392));
#37473=CARTESIAN_POINT('Ctrl Pts',(18.7008270143451,9.68523504562768,-12.0796092025191));
#37474=CARTESIAN_POINT('Ctrl Pts',(18.6938850789891,9.53749998725783,-12.0666882264461));
#37475=CARTESIAN_POINT('Ctrl Pts',(18.6869431436331,9.3903334278217,-12.0473182361383));
#37476=CARTESIAN_POINT('Ctrl Pts',(18.6800012082771,9.244302805183,-12.0215761396486));
#37477=CARTESIAN_POINT('Ctrl Pts',(18.6730576317816,9.0982376595178,-11.9958279574827));
#37478=CARTESIAN_POINT('Ctrl Pts',(18.6661140552862,8.95330931088689,-11.9637047165393));
#37479=CARTESIAN_POINT('Ctrl Pts',(18.6591704787908,8.81007598055744,-11.9253346340039));
#37480=CARTESIAN_POINT('Ctrl Pts',(18.6552746238124,8.72971159148627,-11.9038062073836));
#37481=CARTESIAN_POINT('Ctrl Pts',(18.6513787688341,8.64988059910993,-11.8803121723026));
#37482=CARTESIAN_POINT('Ctrl Pts',(18.6474829138558,8.57067970016459,-11.8548821069951));
#37483=CARTESIAN_POINT('Ctrl Pts',(18.6405493036326,8.4297226661706,-11.8096231941828));
#37484=CARTESIAN_POINT('Ctrl Pts',(18.6336156934094,8.29071373380833,-11.7582135060853));
#37485=CARTESIAN_POINT('Ctrl Pts',(18.6266820831862,8.15419024687287,-11.7008459216614));
#37486=CARTESIAN_POINT('Ctrl Pts',(18.6197497891957,8.01769267669309,-11.6434892275371));
#37487=CARTESIAN_POINT('Ctrl Pts',(18.6128174952052,7.88367991517738,-11.5801770216112));
#37488=CARTESIAN_POINT('Ctrl Pts',(18.6058852012147,7.75266950923779,-11.5111503874492));
#37489=CARTESIAN_POINT('Ctrl Pts',(18.5989526626174,7.62165448058108,-11.4421213176745));
#37490=CARTESIAN_POINT('Ctrl Pts',(18.5920201240202,7.49364231349697,-11.3673775673167));
#37491=CARTESIAN_POINT('Ctrl Pts',(18.5850875854229,7.36912660488231,-11.2872065170139));
#37492=CARTESIAN_POINT('Ctrl Pts',(18.5781554218558,7.24461763220445,-11.2070398037311));
#37493=CARTESIAN_POINT('Ctrl Pts',(18.5712232582886,7.12360501695346,-11.121446557744));
#37494=CARTESIAN_POINT('Ctrl Pts',(18.5642910947215,7.00655398674484,-11.030757893783));
#37495=CARTESIAN_POINT('Ctrl Pts',(18.5573573897854,6.8894769301988,-10.9400490651659));
#37496=CARTESIAN_POINT('Ctrl Pts',(18.5504236848492,6.77636348017962,-10.8442427572896));
#37497=CARTESIAN_POINT('Ctrl Pts',(18.5434899799131,6.6676468407924,-10.7437112207119));
#37498=CARTESIAN_POINT('Ctrl Pts',(18.5393724095913,6.60308562684493,-10.6840107178447));
#37499=CARTESIAN_POINT('Ctrl Pts',(18.5352548392694,6.54007433979697,-10.622644599298));
#37500=CARTESIAN_POINT('Ctrl Pts',(18.5311372689476,6.47869775743707,-10.5596971761229));
#37501=CARTESIAN_POINT('Ctrl Pts',(18.5242037115753,6.37534601797689,-10.4537003051742));
#37502=CARTESIAN_POINT('Ctrl Pts',(18.5172701542029,6.27659580949282,-10.3431810703944));
#37503=CARTESIAN_POINT('Ctrl Pts',(18.5103365968306,6.18283159101337,-10.2285615170703));
#37504=CARTESIAN_POINT('Ctrl Pts',(18.5034043559565,6.089085175867,-10.113963726953));
#37505=CARTESIAN_POINT('Ctrl Pts',(18.4964721150824,6.0003230711042,-9.99526742733144));
#37506=CARTESIAN_POINT('Ctrl Pts',(18.4895398742083,5.91688967035563,-9.87292798562261));
#37507=CARTESIAN_POINT('Ctrl Pts',(18.4826073886049,5.83345332415193,-9.75058422495596));
#37508=CARTESIAN_POINT('Ctrl Pts',(18.4756749030014,5.75534624741186,-9.62459733606426));
#37509=CARTESIAN_POINT('Ctrl Pts',(18.4687424173979,5.68286999196541,-9.49545237815638));
#37510=CARTESIAN_POINT('Ctrl Pts',(18.4618103066269,5.61039765523575,-9.36631440298387));
#37511=CARTESIAN_POINT('Ctrl Pts',(18.4548781958558,5.5435556915652,-9.23401898922316));
#37512=CARTESIAN_POINT('Ctrl Pts',(18.4479460850847,5.48260010633888,-9.09907655369981));
#37513=CARTESIAN_POINT('Ctrl Pts',(18.4410124321748,5.42163096074452,-8.96410409846483));
#37514=CARTESIAN_POINT('Ctrl Pts',(18.434078779265,5.36655094628959,-8.82648374621635));
#37515=CARTESIAN_POINT('Ctrl Pts',(18.4271451263551,5.3175685098331,-8.68674726439385));
#37516=CARTESIAN_POINT('Ctrl Pts',(18.4230272922499,5.28847828134614,-8.6037590245624));
#37517=CARTESIAN_POINT('Ctrl Pts',(18.4189094581446,5.26153778917509,-8.52002479046549));
#37518=CARTESIAN_POINT('Ctrl Pts',(18.4147916240394,5.23678246616714,-8.43565878053404));
#37519=CARTESIAN_POINT('Ctrl Pts',(18.4078580499257,5.19509966341243,-8.29360400912006));
#37520=CARTESIAN_POINT('Ctrl Pts',(18.400924475812,5.15960044824281,-8.1497081866558));
#37521=CARTESIAN_POINT('Ctrl Pts',(18.3939909016982,5.13042688503271,-8.00452426113619));
#37522=CARTESIAN_POINT('Ctrl Pts',(18.3870586444984,5.10125886284241,-7.85936791082228));
#37523=CARTESIAN_POINT('Ctrl Pts',(18.3801263872986,5.07841416062936,-7.71292426949538));
#37524=CARTESIAN_POINT('Ctrl Pts',(18.3731941300988,5.06198383767688,-7.56575696601455));
#37525=CARTESIAN_POINT('Ctrl Pts',(18.3662616289537,5.04555293654322,-7.41858448373312));
#37526=CARTESIAN_POINT('Ctrl Pts',(18.3593291278085,5.03553690634891,-7.27068861649685));
#37527=CARTESIAN_POINT('Ctrl Pts',(18.3523966266634,5.03197504813123,-7.12263916615529));
#37528=CARTESIAN_POINT('Ctrl Pts',(18.3454645008326,5.02841338274678,-6.97459773097103));
#37529=CARTESIAN_POINT('Ctrl Pts',(18.3385323750019,5.0313051971733,-6.82640305983149));
#37530=CARTESIAN_POINT('Ctrl Pts',(18.3316002491711,5.04063767405535,-6.67862603157506));
#37531=CARTESIAN_POINT('Ctrl Pts',(18.3246665820787,5.0499722258837,-6.53081614715388));
#37532=CARTESIAN_POINT('Ctrl Pts',(18.3177329149862,5.06575028063441,-6.38342442119573));
#37533=CARTESIAN_POINT('Ctrl Pts',(18.3107992478938,5.08790700112659,-6.23701832675314));
#37534=CARTESIAN_POINT('Ctrl Pts',(18.3066814916396,5.10106540246934,-6.15007088566497));
#37535=CARTESIAN_POINT('Ctrl Pts',(18.3025637353854,5.11647251715666,-6.06347097260691));
#37536=CARTESIAN_POINT('Ctrl Pts',(18.2984459791312,5.13410616806531,-5.97733609437465));
#37537=CARTESIAN_POINT('Ctrl Pts',(18.2915125307032,5.16379758291008,-5.83230280458991));
#37538=CARTESIAN_POINT('Ctrl Pts',(18.2845790822751,5.19981459172732,-5.68853842305289));
#37539=CARTESIAN_POINT('Ctrl Pts',(18.2776456338471,5.2420237897517,-5.54659802729703));
#37540=CARTESIAN_POINT('Ctrl Pts',(18.2703819990295,5.28624308460534,-5.39789811103834));
#37541=CARTESIAN_POINT('Ctrl Pts',(18.263118364212,5.33725872777692,-5.25120054397503));
#37542=CARTESIAN_POINT('Ctrl Pts',(18.2558547293944,5.3948582910805,-5.10712681667265));
#37543=CARTESIAN_POINT('Ctrl Pts',(18.2489226338069,5.44982879670795,-4.9696291485792));
#37544=CARTESIAN_POINT('Ctrl Pts',(18.2419905382195,5.51079538574318,-4.83452143894434));
#37545=CARTESIAN_POINT('Ctrl Pts',(18.2350584426321,5.57752371529563,-4.70232445643669));
#37546=CARTESIAN_POINT('Ctrl Pts',(18.2281266643766,5.64424899021099,-4.57013352553874));
#37547=CARTESIAN_POINT('Ctrl Pts',(18.2211948861212,5.71673532792395,-4.44085334971581));
#37548=CARTESIAN_POINT('Ctrl Pts',(18.2142631078658,5.79470193918982,-4.31498104811227));
#37549=CARTESIAN_POINT('Ctrl Pts',(18.2073302816422,5.87268033769472,-4.18908971673583));
#37550=CARTESIAN_POINT('Ctrl Pts',(18.2003974554187,5.95614048962211,-4.06660756907976));
#37551=CARTESIAN_POINT('Ctrl Pts',(18.1934646291951,6.04475744071231,-3.94800405892409));
#37552=CARTESIAN_POINT('Ctrl Pts',(18.1924704248088,6.0574655857937,-3.93099568077885));
#37553=CARTESIAN_POINT('Ctrl Pts',(18.1914762204225,6.07027970975569,-3.91406701628419));
#37554=CARTESIAN_POINT('Ctrl Pts',(18.1904820160362,6.08319878352125,-3.89721939777841));
#37555=CARTESIAN_POINT('Ctrl Pts',(19.690497962139,6.08288688923237,-3.89698012451529));
#37556=CARTESIAN_POINT('Ctrl Pts',(19.6530813324665,6.56941784810607,-3.2628032921712));
#37557=CARTESIAN_POINT('Ctrl Pts',(19.5768828211578,7.86759191038278,-2.20936840056837));
#37558=CARTESIAN_POINT('Ctrl Pts',(19.4619024282131,10.3463489318624,-1.69885207129888));
#37559=CARTESIAN_POINT('Ctrl Pts',(19.3455567833049,12.803119455071,-2.41785981379941));
#37560=CARTESIAN_POINT('Ctrl Pts',(19.2292111383967,14.6377971005625,-4.2031950129451));
#37561=CARTESIAN_POINT('Ctrl Pts',(19.1128654934886,15.4225339830853,-6.640033572117));
#37562=CARTESIAN_POINT('Ctrl Pts',(18.9965198485803,14.9749217362807,-9.16055209676269));
#37563=CARTESIAN_POINT('Ctrl Pts',(18.8801742036722,13.399034665446,-11.1780643853626));
#37564=CARTESIAN_POINT('Ctrl Pts',(18.7885520913344,11.5585268032384,-12.0007214198279));
#37565=CARTESIAN_POINT('Ctrl Pts',(18.7357118606328,10.4298968038467,-12.0989142199688));
#37566=CARTESIAN_POINT('Ctrl Pts',(18.7216535115672,10.1295873228123,-12.0987228108905));
#37567=CARTESIAN_POINT('Origin',(26.8463464956315,10.1295,-7.));
#37568=CARTESIAN_POINT('',(21.1904791240421,6.08319878352126,-3.89721939777839));
#37569=CARTESIAN_POINT('',(21.065286535997,6.08319878352127,-3.89721939777838));
#37570=CARTESIAN_POINT('',(26.8463464956315,6.08319878352126,-3.89721939777839));
#37571=CARTESIAN_POINT('',(20.0963464956032,10.1292828156512,-12.0989999953747));
#37572=CARTESIAN_POINT('Ctrl Pts',(21.065286535997,6.08319878352127,-3.89721939777838));
#37573=CARTESIAN_POINT('Ctrl Pts',(21.0585701332919,6.17049443209072,-3.78337812625988));
#37574=CARTESIAN_POINT('Ctrl Pts',(21.0518537305868,6.26254638853162,-3.67329063711811));
#37575=CARTESIAN_POINT('Ctrl Pts',(21.0451373278817,6.35899135444725,-3.5673529814716));
#37576=CARTESIAN_POINT('Ctrl Pts',(21.0384166480659,6.45549773803189,-3.46134786306215));
#37577=CARTESIAN_POINT('Ctrl Pts',(21.0316959682501,6.55640244925519,-3.35949811006252));
#37578=CARTESIAN_POINT('Ctrl Pts',(21.0249752884342,6.6613062164028,-3.26216200465862));
#37579=CARTESIAN_POINT('Ctrl Pts',(21.0182445035305,6.76636771488332,-3.16467954651578));
#37580=CARTESIAN_POINT('Ctrl Pts',(21.0115137186268,6.87544000309704,-3.07172453711754));
#37581=CARTESIAN_POINT('Ctrl Pts',(21.0047829337231,6.98809098247977,-2.98361476142508));
#37582=CARTESIAN_POINT('Ctrl Pts',(21.0004146416252,7.0612016805781,-2.92643135081061));
#37583=CARTESIAN_POINT('Ctrl Pts',(20.9960463495273,7.13581911444332,-2.87128790198545));
#37584=CARTESIAN_POINT('Ctrl Pts',(20.9916780574294,7.21181912996737,-2.81826120607161));
#37585=CARTESIAN_POINT('Ctrl Pts',(20.9851848545906,7.32478857099484,-2.73944021958085));
#37586=CARTESIAN_POINT('Ctrl Pts',(20.9786916517519,7.4411732082542,-2.66504792986056));
#37587=CARTESIAN_POINT('Ctrl Pts',(20.9721984489131,7.5605842685465,-2.59540320066743));
#37588=CARTESIAN_POINT('Ctrl Pts',(20.9657137060064,7.679839749308,-2.52584921092728));
#37589=CARTESIAN_POINT('Ctrl Pts',(20.9592289630997,7.80211347051069,-2.46103068201192));
#37590=CARTESIAN_POINT('Ctrl Pts',(20.9527442201929,7.92698482267712,-2.40122539216561));
#37591=CARTESIAN_POINT('Ctrl Pts',(20.9462662847788,8.05172508856592,-2.3414828841559));
#37592=CARTESIAN_POINT('Ctrl Pts',(20.9397883493647,8.17905720344193,-2.28674332075737));
#37593=CARTESIAN_POINT('Ctrl Pts',(20.9333104139506,8.30853331594396,-2.23724015558648));
#37594=CARTESIAN_POINT('Ctrl Pts',(20.9268376417297,8.43790623041245,-2.18777644656854));
#37595=CARTESIAN_POINT('Ctrl Pts',(20.9203648695089,8.56941937043644,-2.14354097624662));
#37596=CARTESIAN_POINT('Ctrl Pts',(20.9138920972881,8.70260256867513,-2.10472015912487));
#37597=CARTESIAN_POINT('Ctrl Pts',(20.9074222385478,8.83572581939206,-2.06591681576715));
#37598=CARTESIAN_POINT('Ctrl Pts',(20.9009523798075,8.97051725008503,-2.03252339372634));
#37599=CARTESIAN_POINT('Ctrl Pts',(20.8944825210672,9.10648943524987,-2.00467714913144));
#37600=CARTESIAN_POINT('Ctrl Pts',(20.8880140950405,9.24243151014331,-1.97683707092991));
#37601=CARTESIAN_POINT('Ctrl Pts',(20.8815456690139,9.37955342700083,-1.95454180910603));
#37602=CARTESIAN_POINT('Ctrl Pts',(20.8750772429872,9.51735593402374,-1.9378778518797));
#37603=CARTESIAN_POINT('Ctrl Pts',(20.8686087712673,9.65515941448958,-1.92121377693845));
#37604=CARTESIAN_POINT('Ctrl Pts',(20.8621402995473,9.79364309633691,-1.91018113416165));
#37605=CARTESIAN_POINT('Ctrl Pts',(20.8556718278274,9.93230148099877,-1.90481465066248));
#37606=CARTESIAN_POINT('Ctrl Pts',(20.8492018320788,10.0709925347921,-1.89944690277274));
#37607=CARTESIAN_POINT('Ctrl Pts',(20.8427318363303,10.2098579723932,-1.89974798431355));
#37608=CARTESIAN_POINT('Ctrl Pts',(20.8362618405817,10.3483917041282,-1.90570049743207));
#37609=CARTESIAN_POINT('Ctrl Pts',(20.8297845845165,10.487080891723,-1.91165969017319));
#37610=CARTESIAN_POINT('Ctrl Pts',(20.8233073284513,10.6254372286393,-1.92328296238101));
#37611=CARTESIAN_POINT('Ctrl Pts',(20.8168300723862,10.7629587075552,-1.94050090761719));
#37612=CARTESIAN_POINT('Ctrl Pts',(20.8103491685815,10.9005576332364,-1.95772854933259));
#37613=CARTESIAN_POINT('Ctrl Pts',(20.8038682647768,11.0373203698773,-1.98055707009135));
#37614=CARTESIAN_POINT('Ctrl Pts',(20.7973873609722,11.1727557922057,-2.00886602543778));
#37615=CARTESIAN_POINT('Ctrl Pts',(20.7908954455443,11.3084213311775,-2.03722308017853));
#37616=CARTESIAN_POINT('Ctrl Pts',(20.7844035301165,11.4427546621825,-2.07107907258745));
#37617=CARTESIAN_POINT('Ctrl Pts',(20.7779116146887,11.5752797123965,-2.11026360391251));
#37618=CARTESIAN_POINT('Ctrl Pts',(20.7716033323302,11.7040561029136,-2.14833974498919));
#37619=CARTESIAN_POINT('Ctrl Pts',(20.7652950499716,11.8311248479606,-2.19144685620594));
#37620=CARTESIAN_POINT('Ctrl Pts',(20.758986767613,11.956069933585,-2.23938624989138));
#37621=CARTESIAN_POINT('Ctrl Pts',(20.752255350081,12.089395852133,-2.29054123262481));
#37622=CARTESIAN_POINT('Ctrl Pts',(20.7455239325489,12.2207429681633,-2.34736702175228));
#37623=CARTESIAN_POINT('Ctrl Pts',(20.7387925150168,12.3496051713782,-2.40969129273208));
#37624=CARTESIAN_POINT('Ctrl Pts',(20.7320693455013,12.4783094795322,-2.47193919768429));
#37625=CARTESIAN_POINT('Ctrl Pts',(20.7253461759858,12.604534607748,-2.53967200821282));
#37626=CARTESIAN_POINT('Ctrl Pts',(20.7186230064702,12.7277927942082,-2.61266874335141));
#37627=CARTESIAN_POINT('Ctrl Pts',(20.7119067023597,12.8509251148298,-2.68559093743474));
#37628=CARTESIAN_POINT('Ctrl Pts',(20.7051903982492,12.9710962113983,-2.7637661629336));
#37629=CARTESIAN_POINT('Ctrl Pts',(20.6984740941386,13.0878414666366,-2.84692682862695));
#37630=CARTESIAN_POINT('Ctrl Pts',(20.691763278558,13.2044913182398,-2.93001953584278));
#37631=CARTESIAN_POINT('Ctrl Pts',(20.6850524629774,13.3177206051619,-3.01808935397584));
#37632=CARTESIAN_POINT('Ctrl Pts',(20.6783416473968,13.427092417135,-3.11082460533681));
#37633=CARTESIAN_POINT('Ctrl Pts',(20.6716350714244,13.5363951326426,-3.20350127050457));
#37634=CARTESIAN_POINT('Ctrl Pts',(20.6649284954521,13.6418449478012,-3.30083725726319));
#37635=CARTESIAN_POINT('Ctrl Pts',(20.6582219194797,13.7430369628603,-3.40247979602026));
#37636=CARTESIAN_POINT('Ctrl Pts',(20.6515176619563,13.8441939960568,-3.50408719716967));
#37637=CARTESIAN_POINT('Ctrl Pts',(20.6448134044329,13.9410958999718,-3.60999792371146));
#37638=CARTESIAN_POINT('Ctrl Pts',(20.6381091469095,14.0333736471028,-3.71982141531038));
#37639=CARTESIAN_POINT('Ctrl Pts',(20.6314059678938,14.1256365495977,-3.82962723970549));
#37640=CARTESIAN_POINT('Ctrl Pts',(20.6247027888781,14.2132765396375,-3.94334429217381));
#37641=CARTESIAN_POINT('Ctrl Pts',(20.6179996098624,14.2959640876569,-4.060548009192));
#37642=CARTESIAN_POINT('Ctrl Pts',(20.6112962704155,14.378653614687,-4.17775453131697));
#37643=CARTESIAN_POINT('Ctrl Pts',(20.6045929309686,14.456390251492,-4.29844758149486));
#37644=CARTESIAN_POINT('Ctrl Pts',(20.5978895915217,14.5288871829675,-4.42217273380445));
#37645=CARTESIAN_POINT('Ctrl Pts',(20.5911823410669,14.6014264121778,-4.54597007253031));
#37646=CARTESIAN_POINT('Ctrl Pts',(20.5844750906121,14.668719640705,-4.67280272880459));
#37647=CARTESIAN_POINT('Ctrl Pts',(20.5777678401573,14.7305252782473,-4.80219032013015));
#37648=CARTESIAN_POINT('Ctrl Pts',(20.5710585028671,14.7923501454557,-4.93161816798048));
#37649=CARTESIAN_POINT('Ctrl Pts',(20.564349165577,14.8486838674656,-5.06360219779874));
#37650=CARTESIAN_POINT('Ctrl Pts',(20.5576398282869,14.8993327590442,-5.19764142004176));
#37651=CARTESIAN_POINT('Ctrl Pts',(20.5509240694714,14.9500301268172,-5.33180893159575));
#37652=CARTESIAN_POINT('Ctrl Pts',(20.544208310656,14.9950316728671,-5.4680352158438));
#37653=CARTESIAN_POINT('Ctrl Pts',(20.5374925518406,15.0341932052633,-5.60580289691735));
#37654=CARTESIAN_POINT('Ctrl Pts',(20.5337601938259,15.055957664548,-5.68236882531709));
#37655=CARTESIAN_POINT('Ctrl Pts',(20.5300278358113,15.0759192163065,-5.75941061027489));
#37656=CARTESIAN_POINT('Ctrl Pts',(20.5262954777967,15.0940599329618,-5.83683807144917));
#37657=CARTESIAN_POINT('Ctrl Pts',(20.5195531565522,15.1268302456745,-5.97670697318204));
#37658=CARTESIAN_POINT('Ctrl Pts',(20.5128108353077,15.1537122172889,-6.11807599491532));
#37659=CARTESIAN_POINT('Ctrl Pts',(20.5060685140632,15.174579088646,-6.26042039691011));
#37660=CARTESIAN_POINT('Ctrl Pts',(20.4993310938359,15.1954307918007,-6.40266132825656));
#37661=CARTESIAN_POINT('Ctrl Pts',(20.4925936736085,15.210276051231,-6.54587586687352));
#37662=CARTESIAN_POINT('Ctrl Pts',(20.4858562533812,15.2190391491384,-6.68952898784726));
#37663=CARTESIAN_POINT('Ctrl Pts',(20.4791225787158,15.2277973753404,-6.83310224714431));
#37664=CARTESIAN_POINT('Ctrl Pts',(20.4723889040505,15.2304801549966,-6.97711323862747));
#37665=CARTESIAN_POINT('Ctrl Pts',(20.4656552293852,15.2270636067672,-7.12102179540484));
#37666=CARTESIAN_POINT('Ctrl Pts',(20.4589238948687,15.2236482458881,-7.26488033975003));
#37667=CARTESIAN_POINT('Ctrl Pts',(20.4521925603523,15.2141377896593,-7.40863615508435));
#37668=CARTESIAN_POINT('Ctrl Pts',(20.4454612258358,15.1985604617483,-7.55174906899793));
#37669=CARTESIAN_POINT('Ctrl Pts',(20.4387300007792,15.182983387144,-7.69485965571773));
#37670=CARTESIAN_POINT('Ctrl Pts',(20.4319987757227,15.161339670661,-7.83732699762328));
#37671=CARTESIAN_POINT('Ctrl Pts',(20.4252675506661,15.1337094284332,-7.97861585741328));
#37672=CARTESIAN_POINT('Ctrl Pts',(20.4201616447402,15.1127507743489,-8.08578916099401));
#37673=CARTESIAN_POINT('Ctrl Pts',(20.4150557388143,15.0883486417902,-8.19228444747344));
#37674=CARTESIAN_POINT('Ctrl Pts',(20.4099498328885,15.0605576408463,-8.2978719284471));
#37675=CARTESIAN_POINT('Ctrl Pts',(20.4026904401681,15.0210453989695,-8.44799239714914));
#37676=CARTESIAN_POINT('Ctrl Pts',(20.3954310474478,14.9746959459559,-8.59622252503325));
#37677=CARTESIAN_POINT('Ctrl Pts',(20.3881716547275,14.9217167822243,-8.74196995156864));
#37678=CARTESIAN_POINT('Ctrl Pts',(20.3809048355569,14.8686834201407,-8.88786647955733));
#37679=CARTESIAN_POINT('Ctrl Pts',(20.3736380163864,14.8090068857943,-9.03127499398435));
#37680=CARTESIAN_POINT('Ctrl Pts',(20.3663711972158,14.7429431237293,-9.17162232999089));
#37681=CARTESIAN_POINT('Ctrl Pts',(20.3590963867037,14.6768067111584,-9.31212400635949));
#37682=CARTESIAN_POINT('Ctrl Pts',(20.3518215761916,14.6042691365757,-9.44955754437085));
#37683=CARTESIAN_POINT('Ctrl Pts',(20.3445467656795,14.5256333395251,-9.58337234271712));
#37684=CARTESIAN_POINT('Ctrl Pts',(20.337269635131,14.4469724644459,-9.71722981642851));
#37685=CARTESIAN_POINT('Ctrl Pts',(20.3299925045826,14.3622096156487,-9.84746602947761));
#37686=CARTESIAN_POINT('Ctrl Pts',(20.3227153740341,14.2716922118622,-9.97355757973308));
#37687=CARTESIAN_POINT('Ctrl Pts',(20.3154369289258,14.1811584567754,-10.0996719074956));
#37688=CARTESIAN_POINT('Ctrl Pts',(20.3081584838175,14.0848682185007,-10.2216398712836));
#37689=CARTESIAN_POINT('Ctrl Pts',(20.3008800387091,13.983211124939,-10.3389686379961));
#37690=CARTESIAN_POINT('Ctrl Pts',(20.2984547551328,13.9493375055381,-10.3780642864073));
#37691=CARTESIAN_POINT('Ctrl Pts',(20.2960294715565,13.9148683294575,-10.4166451029411));
#37692=CARTESIAN_POINT('Ctrl Pts',(20.2936041879802,13.8798190021703,-10.4546936741136));
#37693=CARTESIAN_POINT('Ctrl Pts',(20.2868777084082,13.7826103349796,-10.5602206892792));
#37694=CARTESIAN_POINT('Ctrl Pts',(20.2801512288361,13.6808807511221,-10.6617110339456));
#37695=CARTESIAN_POINT('Ctrl Pts',(20.2734247492641,13.5749966495666,-10.7587702560579));
#37696=CARTESIAN_POINT('Ctrl Pts',(20.2667018516651,13.469168933226,-10.8557777923645));
#37697=CARTESIAN_POINT('Ctrl Pts',(20.2599789540661,13.3591913769016,-10.9483586585881));
#37698=CARTESIAN_POINT('Ctrl Pts',(20.2532560564671,13.2454670553348,-11.0361553872551));
#37699=CARTESIAN_POINT('Ctrl Pts',(20.2465348108106,13.1317706779763,-11.1239305426118));
#37700=CARTESIAN_POINT('Ctrl Pts',(20.2398135651542,13.0143296577915,-11.2069236743742));
#37701=CARTESIAN_POINT('Ctrl Pts',(20.2330923194978,12.8935800092736,-11.2848176976779));
#37702=CARTESIAN_POINT('Ctrl Pts',(20.2263722417576,12.7728513428002,-11.3626981857384));
#37703=CARTESIAN_POINT('Ctrl Pts',(20.2196521640174,12.6488155039475,-11.4354811335248));
#37704=CARTESIAN_POINT('Ctrl Pts',(20.2129320862773,12.5219371004029,-11.5028930389935));
#37705=CARTESIAN_POINT('Ctrl Pts',(20.2062101801347,12.3950241757137,-11.5703232859298));
#37706=CARTESIAN_POINT('Ctrl Pts',(20.1994882739921,12.2652674652435,-11.6323793963712));
#37707=CARTESIAN_POINT('Ctrl Pts',(20.1927663678496,12.1331560519276,-11.6888339089345));
#37708=CARTESIAN_POINT('Ctrl Pts',(20.1875970929237,12.0315598377311,-11.7322485133716));
#37709=CARTESIAN_POINT('Ctrl Pts',(20.1824278179979,11.9285716059888,-11.7723513056034));
#37710=CARTESIAN_POINT('Ctrl Pts',(20.1772585430721,11.8244215995656,-11.8090583040057));
#37711=CARTESIAN_POINT('Ctrl Pts',(20.1702029153173,11.6822655551441,-11.8591602855097));
#37712=CARTESIAN_POINT('Ctrl Pts',(20.1631472875625,11.5378982969924,-11.9029508158294));
#37713=CARTESIAN_POINT('Ctrl Pts',(20.1560916598077,11.3918866567047,-11.9402612207224));
#37714=CARTESIAN_POINT('Ctrl Pts',(20.1490358127607,11.245870478308,-11.9775727852401));
#37715=CARTESIAN_POINT('Ctrl Pts',(20.1419799657137,11.0982101122984,-12.0084037507865));
#37716=CARTESIAN_POINT('Ctrl Pts',(20.1349241186668,10.9494848386558,-12.0326360750977));
#37717=CARTESIAN_POINT('Ctrl Pts',(20.1278666858757,10.8007261402202,-12.0568738454262));
#37718=CARTESIAN_POINT('Ctrl Pts',(20.1208092530846,10.6509023569821,-12.0745099618943));
#37719=CARTESIAN_POINT('Ctrl Pts',(20.1137518202935,10.5006010709216,-12.0854778531777));
#37720=CARTESIAN_POINT('Ctrl Pts',(20.1079500454062,10.3770413782099,-12.0944943380808));
#37721=CARTESIAN_POINT('Ctrl Pts',(20.1021482705188,10.2531592030081,-12.0990052716912));
#37722=CARTESIAN_POINT('Ctrl Pts',(20.0963464956315,10.1292828162553,-12.0989999953747));
#37723=CARTESIAN_POINT('Ctrl Pts',(20.0963464956032,10.1292828156512,-12.0989999953747));
#37724=CARTESIAN_POINT('Ctrl Pts',(20.0890161304489,9.9727687890773,-12.0989933288916));
#37725=CARTESIAN_POINT('Ctrl Pts',(20.0816857652947,9.81628384987453,-12.0917760164965));
#37726=CARTESIAN_POINT('Ctrl Pts',(20.0743554001404,9.66046609801297,-12.0773820221436));
#37727=CARTESIAN_POINT('Ctrl Pts',(20.0698745661482,9.56521934502955,-12.0685834019081));
#37728=CARTESIAN_POINT('Ctrl Pts',(20.065393732156,9.4702218440322,-12.0571042223294));
#37729=CARTESIAN_POINT('Ctrl Pts',(20.0609128981638,9.37561849205956,-12.0429617956103));
#37730=CARTESIAN_POINT('Ctrl Pts',(20.0540297945509,9.23029628755551,-12.0212373156105));
#37731=CARTESIAN_POINT('Ctrl Pts',(20.0471466909379,9.0858734579511,-11.9932209241342));
#37732=CARTESIAN_POINT('Ctrl Pts',(20.040263587325,8.94290407468458,-11.9590111020268));
#37733=CARTESIAN_POINT('Ctrl Pts',(20.0333824104595,8.79997471201355,-11.9248108560777));
#37734=CARTESIAN_POINT('Ctrl Pts',(20.0265012335941,8.65849831506874,-11.8844207161138));
#37735=CARTESIAN_POINT('Ctrl Pts',(20.0196200567286,8.51901756866879,-11.8379900101564));
#37736=CARTESIAN_POINT('Ctrl Pts',(20.0127390888202,8.37954105780559,-11.7915607141354));
#37737=CARTESIAN_POINT('Ctrl Pts',(20.0058581209118,8.24206040107134,-11.7390913207874));
#37738=CARTESIAN_POINT('Ctrl Pts',(19.9989771530033,8.10710237471126,-11.6807807944003));
#37739=CARTESIAN_POINT('Ctrl Pts',(19.9920967087737,7.97215461938547,-11.6224747057589));
#37740=CARTESIAN_POINT('Ctrl Pts',(19.985216264544,7.83972942282541,-11.5583285083938));
#37741=CARTESIAN_POINT('Ctrl Pts',(19.9783358203144,7.71033280260142,-11.4885889844171));
#37742=CARTESIAN_POINT('Ctrl Pts',(19.9714536339439,7.58090341892158,-11.4188318022682));
#37743=CARTESIAN_POINT('Ctrl Pts',(19.9645714475735,7.45450444365356,-11.3434786251353));
#37744=CARTESIAN_POINT('Ctrl Pts',(19.957689261203,7.33161704422618,-11.2628220659312));
#37745=CARTESIAN_POINT('Ctrl Pts',(19.9533152585539,7.25351543788963,-11.2115604486721));
#37746=CARTESIAN_POINT('Ctrl Pts',(19.9489412559048,7.17683173753798,-11.1581575511211));
#37747=CARTESIAN_POINT('Ctrl Pts',(19.9445672532557,7.10168335770222,-11.1026975736245));
#37748=CARTESIAN_POINT('Ctrl Pts',(19.9376178748488,6.9822882475402,-11.0145832305441));
#37749=CARTESIAN_POINT('Ctrl Pts',(19.930668496442,6.8667251055417,-10.921240950437));
#37750=CARTESIAN_POINT('Ctrl Pts',(19.9237191180351,6.75544289250122,-10.8230275483361));
#37751=CARTESIAN_POINT('Ctrl Pts',(19.9167708710451,6.64417879713505,-10.7248301361979));
#37752=CARTESIAN_POINT('Ctrl Pts',(19.9098226240551,6.53719448530056,-10.6217634011466));
#37753=CARTESIAN_POINT('Ctrl Pts',(19.9028743770652,6.43490468373816,-10.5142234489366));
#37754=CARTESIAN_POINT('Ctrl Pts',(19.8959257674772,6.33260954412695,-10.4066778846959));
#37755=CARTESIAN_POINT('Ctrl Pts',(19.8889771578891,6.23500963255852,-10.2946588716185));
#37756=CARTESIAN_POINT('Ctrl Pts',(19.8820285483011,6.14248214411779,-10.1785986876101));
#37757=CARTESIAN_POINT('Ctrl Pts',(19.8750802871826,6.04995929588631,-10.0625443239643));
#37758=CARTESIAN_POINT('Ctrl Pts',(19.868132026064,5.96250856499122,-9.94244945163858));
#37759=CARTESIAN_POINT('Ctrl Pts',(19.8611837649454,5.88046626630638,-9.8187786947424));
#37760=CARTESIAN_POINT('Ctrl Pts',(19.8542340645085,5.79840697272408,-9.6950823196972));
#37761=CARTESIAN_POINT('Ctrl Pts',(19.8472843640716,5.72175853102108,-9.56780885290348));
#37762=CARTESIAN_POINT('Ctrl Pts',(19.8403346636347,5.65081375603784,-9.43745164631919));
#37763=CARTESIAN_POINT('Ctrl Pts',(19.8362969785389,5.60959576928118,-9.36171581354087));
#37764=CARTESIAN_POINT('Ctrl Pts',(19.8322592934432,5.57030220177107,-9.28493958658977));
#37765=CARTESIAN_POINT('Ctrl Pts',(19.8282216083474,5.53298336328829,-9.20722355198392));
#37766=CARTESIAN_POINT('Ctrl Pts',(19.821289621329,5.46891355651218,-9.07379894599301));
#37767=CARTESIAN_POINT('Ctrl Pts',(19.8143576343105,5.41064597993131,-8.93755962820844));
#37768=CARTESIAN_POINT('Ctrl Pts',(19.807425647292,5.35841008944348,-8.79902808910417));
#37769=CARTESIAN_POINT('Ctrl Pts',(19.800494976297,5.30618411583254,-8.66052284992904));
#37770=CARTESIAN_POINT('Ctrl Pts',(19.7935643053021,5.25998766035838,-8.51972656710486));
#37771=CARTESIAN_POINT('Ctrl Pts',(19.7866336343072,5.22000157021081,-8.37718051391147));
#37772=CARTESIAN_POINT('Ctrl Pts',(19.7797027024116,5.18001397481245,-8.23462909466308));
#37773=CARTESIAN_POINT('Ctrl Pts',(19.772771770516,5.14623730510447,-8.09032809093049));
#37774=CARTESIAN_POINT('Ctrl Pts',(19.7658408386203,5.11880232749438,-7.94483323118251));
#37775=CARTESIAN_POINT('Ctrl Pts',(19.7589102686247,5.09136878240709,-7.7993459684775));
#37776=CARTESIAN_POINT('Ctrl Pts',(19.7519796986291,5.07027632712535,-7.65266529985237));
#37777=CARTESIAN_POINT('Ctrl Pts',(19.7450491286335,5.05560446738238,-7.50535643271154));
#37778=CARTESIAN_POINT('Ctrl Pts',(19.73811698291,5.04092927185914,-7.35801407356488));
#37779=CARTESIAN_POINT('Ctrl Pts',(19.7311848371864,5.03267762147763,-7.21004355990087));
#37780=CARTESIAN_POINT('Ctrl Pts',(19.7242526914629,5.03087713469774,-7.06201513861103));
#37781=CARTESIAN_POINT('Ctrl Pts',(19.720127115455,5.02980559850131,-6.97391795662521));
#37782=CARTESIAN_POINT('Ctrl Pts',(19.7160015394472,5.03101799301621,-6.88580032960711));
#37783=CARTESIAN_POINT('Ctrl Pts',(19.7118759634393,5.03451137520289,-6.7977825101827));
#37784=CARTESIAN_POINT('Ctrl Pts',(19.7049446719573,5.04038053144858,-6.64990566562309));
#37785=CARTESIAN_POINT('Ctrl Pts',(19.6980133804754,5.05269303632925,-6.50225813648039));
#37786=CARTESIAN_POINT('Ctrl Pts',(19.6910820889935,5.07140714354957,-6.35540892379343));
#37787=CARTESIAN_POINT('Ctrl Pts',(19.684152155773,5.09011758353832,-6.20858848779685));
#37788=CARTESIAN_POINT('Ctrl Pts',(19.6772222225525,5.11522708127018,-6.06256638434076));
#37789=CARTESIAN_POINT('Ctrl Pts',(19.6702922893321,5.1466421432545,-5.91790546648196));
#37790=CARTESIAN_POINT('Ctrl Pts',(19.6633621517524,5.17805813164832,-5.77324028266789));
#37791=CARTESIAN_POINT('Ctrl Pts',(19.6564320141728,5.21577998959384,-5.62993668900659));
#37792=CARTESIAN_POINT('Ctrl Pts',(19.6495018765932,5.25966320185877,-5.48854687156048));
#37793=CARTESIAN_POINT('Ctrl Pts',(19.6425721311451,5.30354393105683,-5.34716505444877));
#37794=CARTESIAN_POINT('Ctrl Pts',(19.6356423856971,5.3535852180655,-5.20769711279107));
#37795=CARTESIAN_POINT('Ctrl Pts',(19.6287126402491,5.40959281113337,-5.07067962005138));
#37796=CARTESIAN_POINT('Ctrl Pts',(19.6217813588474,5.46561281808687,-4.93363175786727));
#37797=CARTESIAN_POINT('Ctrl Pts',(19.6148500774458,5.52760164817825,-4.79903573639779));
#37798=CARTESIAN_POINT('Ctrl Pts',(19.6079187960441,5.59531683860077,-4.66740829571833));
#37799=CARTESIAN_POINT('Ctrl Pts',(19.6037893035398,5.63565993752784,-4.58898779911019));
#37800=CARTESIAN_POINT('Ctrl Pts',(19.5996598110354,5.6780346941485,-4.51162059036813));
#37801=CARTESIAN_POINT('Ctrl Pts',(19.5955303185311,5.72238203724709,-4.43541187275996));
#37802=CARTESIAN_POINT('Ctrl Pts',(19.5885944590229,5.79686744700874,-4.30741237692011));
#37803=CARTESIAN_POINT('Ctrl Pts',(19.5816585995147,5.87694546042748,-4.18263866391877));
#37804=CARTESIAN_POINT('Ctrl Pts',(19.5747227400066,5.96231200227857,-4.06157436853568));
#37805=CARTESIAN_POINT('Ctrl Pts',(19.5715384419151,6.00150433539447,-4.00599296521056));
#37806=CARTESIAN_POINT('Ctrl Pts',(19.5683541438237,6.04181076065445,-3.95119305197544));
#37807=CARTESIAN_POINT('Ctrl Pts',(19.5651698457322,6.08319878352126,-3.8972193977784));
#37808=CARTESIAN_POINT('',(20.2216535043684,10.1337426824875,-12.0989982349129));
#37809=CARTESIAN_POINT('Ctrl Pts',(20.2216531628861,10.1337360354165,-12.0997534730252));
#37810=CARTESIAN_POINT('Ctrl Pts',(20.1623123261755,8.86943546207591,-12.0878187862941));
#37811=CARTESIAN_POINT('Ctrl Pts',(20.0641896078287,6.76854703791684,-11.2892745934799));
#37812=CARTESIAN_POINT('Ctrl Pts',(19.9272850078459,5.12804044036981,-8.75245917967931));
#37813=CARTESIAN_POINT('Ctrl Pts',(19.8109393629377,4.88151594588123,-6.21192105474875));
#37814=CARTESIAN_POINT('Ctrl Pts',(19.7320103477021,5.54900739211662,-4.60515275155534));
#37815=CARTESIAN_POINT('Ctrl Pts',(19.6918632141025,6.06513442588355,-3.92011986674037));
#37816=CARTESIAN_POINT('Ctrl Pts',(19.690497962139,6.08288688923237,-3.89698012451529));
#37817=CARTESIAN_POINT('Ctrl Pts',(21.1904791240421,6.08319878352127,-3.89721939777839));
#37818=CARTESIAN_POINT('Ctrl Pts',(21.1834167056448,6.17494656980835,-3.77757214363582));
#37819=CARTESIAN_POINT('Ctrl Pts',(21.1763542872475,6.27200884096288,-3.66199150568125));
#37820=CARTESIAN_POINT('Ctrl Pts',(21.1692918688503,6.37400656717798,-3.55093199892628));
#37821=CARTESIAN_POINT('Ctrl Pts',(21.1622298870913,6.47599798732141,-3.43987935849309));
#37822=CARTESIAN_POINT('Ctrl Pts',(21.1551679053324,6.58292404919854,-3.33334751629621));
#37823=CARTESIAN_POINT('Ctrl Pts',(21.1481059235734,6.69436714454001,-3.23175594403185));
#37824=CARTESIAN_POINT('Ctrl Pts',(21.1410452118414,6.80579019795256,-3.13018264199826));
#37825=CARTESIAN_POINT('Ctrl Pts',(21.1339845001094,6.92172843775375,-3.03354804002583));
#37826=CARTESIAN_POINT('Ctrl Pts',(21.1269237883774,7.04172903905915,-2.9422331889609));
#37827=CARTESIAN_POINT('Ctrl Pts',(21.1198640177282,7.16171364615532,-2.85093050874193));
#37828=CARTESIAN_POINT('Ctrl Pts',(21.112804247079,7.28575929258829,-2.76494634862895));
#37829=CARTESIAN_POINT('Ctrl Pts',(21.1057444764298,7.41338136355489,-2.68462046249052));
#37830=CARTESIAN_POINT('Ctrl Pts',(21.1007434699292,7.50378639769025,-2.62771914108665));
#37831=CARTESIAN_POINT('Ctrl Pts',(21.0957424634285,7.5959854190011,-2.57365630587753));
#37832=CARTESIAN_POINT('Ctrl Pts',(21.0907414569279,7.68979747601854,-2.52253949269471));
#37833=CARTESIAN_POINT('Ctrl Pts',(21.0840196099996,7.81589015100785,-2.45383344449506));
#37834=CARTESIAN_POINT('Ctrl Pts',(21.0772977630712,7.9449362626361,-2.39043095335399));
#37835=CARTESIAN_POINT('Ctrl Pts',(21.0705759161429,8.07645702253597,-2.33257934907452));
#37836=CARTESIAN_POINT('Ctrl Pts',(21.0638557183066,8.20794551603063,-2.27474193771263));
#37837=CARTESIAN_POINT('Ctrl Pts',(21.0571355204702,8.34190711156151,-2.22245284749552));
#37838=CARTESIAN_POINT('Ctrl Pts',(21.0504153226339,8.47784123377184,-2.17591207377585));
#37839=CARTESIAN_POINT('Ctrl Pts',(21.0436938073277,8.61380200536455,-2.12936217590945));
#37840=CARTESIAN_POINT('Ctrl Pts',(21.0369722920214,8.75173573007874,-2.08856297103887));
#37841=CARTESIAN_POINT('Ctrl Pts',(21.0302507767151,8.89112448377531,-2.05366528823461));
#37842=CARTESIAN_POINT('Ctrl Pts',(21.0235287760831,9.03052330201039,-2.01876508564978));
#37843=CARTESIAN_POINT('Ctrl Pts',(21.0168067754511,9.17137700030015,-1.98976733838324));
#37844=CARTESIAN_POINT('Ctrl Pts',(21.0100847748191,9.31315578902763,-1.96677209643634));
#37845=CARTESIAN_POINT('Ctrl Pts',(21.0033583161372,9.45502860584993,-1.94376160397975));
#37846=CARTESIAN_POINT('Ctrl Pts',(20.9966318574553,9.59782737480171,-1.92676162587731));
#37847=CARTESIAN_POINT('Ctrl Pts',(20.9899053987734,9.74101492534841,-1.91582058275154));
#37848=CARTESIAN_POINT('Ctrl Pts',(20.9847355365222,9.85106687800675,-1.90741144972626));
#37849=CARTESIAN_POINT('Ctrl Pts',(20.9795656742709,9.96134831898086,-1.90258042790854));
#37850=CARTESIAN_POINT('Ctrl Pts',(20.9743958120197,10.071614880693,-1.90132857373974));
#37851=CARTESIAN_POINT('Ctrl Pts',(20.9671175717702,10.2268504534471,-1.89956618724759));
#37852=CARTESIAN_POINT('Ctrl Pts',(20.9598393315207,10.38215201505,-1.90489782475772));
#37853=CARTESIAN_POINT('Ctrl Pts',(20.9525610912711,10.5368917561104,-1.91730062299045));
#37854=CARTESIAN_POINT('Ctrl Pts',(20.9452837330259,10.6916127452311,-1.92970191820577));
#37855=CARTESIAN_POINT('Ctrl Pts',(20.9380063747807,10.8457717972154,-1.94917264147978));
#37856=CARTESIAN_POINT('Ctrl Pts',(20.9307290165355,10.998745255065,-1.97563798213674));
#37857=CARTESIAN_POINT('Ctrl Pts',(20.9234560005045,11.1516274375505,-2.00208753159934));
#37858=CARTESIAN_POINT('Ctrl Pts',(20.9161829844736,11.3033251896582,-2.03552331724142));
#37859=CARTESIAN_POINT('Ctrl Pts',(20.9089099684426,11.4532236629269,-2.07581918851396));
#37860=CARTESIAN_POINT('Ctrl Pts',(20.9016417943633,11.6030223424974,-2.11608823313558));
#37861=CARTESIAN_POINT('Ctrl Pts',(20.894373620284,11.7510238897501,-2.16320818147162));
#37862=CARTESIAN_POINT('Ctrl Pts',(20.8871054462047,11.8966261080614,-2.21700237108486));
#37863=CARTESIAN_POINT('Ctrl Pts',(20.8798462532636,12.0420484086068,-2.27073008828768));
#37864=CARTESIAN_POINT('Ctrl Pts',(20.8725870603225,12.1850770620086,-2.33111549332836));
#37865=CARTESIAN_POINT('Ctrl Pts',(20.8653278673814,12.3251271892484,-2.39793282906112));
#37866=CARTESIAN_POINT('Ctrl Pts',(20.8629019672915,12.3719295843671,-2.42026205795495));
#37867=CARTESIAN_POINT('Ctrl Pts',(20.8604760672015,12.4183994834494,-2.44330918750438));
#37868=CARTESIAN_POINT('Ctrl Pts',(20.8580501671115,12.4645155072712,-2.46706457350171));
#37869=CARTESIAN_POINT('Ctrl Pts',(20.851319308004,12.5924682041796,-2.53297584365391));
#37870=CARTESIAN_POINT('Ctrl Pts',(20.8445884488965,12.7176517637429,-2.60432077926021));
#37871=CARTESIAN_POINT('Ctrl Pts',(20.8378575897889,12.8395943566171,-2.68083462018041));
#37872=CARTESIAN_POINT('Ctrl Pts',(20.8311269491109,12.9615329922165,-2.75734597807738));
#37873=CARTESIAN_POINT('Ctrl Pts',(20.8243963084329,13.0802305615075,-2.8390257118703));
#37874=CARTESIAN_POINT('Ctrl Pts',(20.8176656677548,13.1952429162414,-2.92556490154576));
#37875=CARTESIAN_POINT('Ctrl Pts',(20.8109315848184,13.3103140918602,-3.01214835004661));
#37876=CARTESIAN_POINT('Ctrl Pts',(20.804197501882,13.4216959931946,-3.10359600184866));
#37877=CARTESIAN_POINT('Ctrl Pts',(20.7974634189456,13.52897595819,-3.19955736661001));
#37878=CARTESIAN_POINT('Ctrl Pts',(20.790727670196,13.6362824610811,-3.29554246937953));
#37879=CARTESIAN_POINT('Ctrl Pts',(20.7839919214463,13.7394847375183,-3.3960432610415));
#37880=CARTESIAN_POINT('Ctrl Pts',(20.7772561726966,13.8382061214154,-3.5006715065636));
#37881=CARTESIAN_POINT('Ctrl Pts',(20.7705141740967,13.9370191052046,-3.60539683273453));
#37882=CARTESIAN_POINT('Ctrl Pts',(20.7637721754969,14.0313426428299,-3.71425699380575));
#37883=CARTESIAN_POINT('Ctrl Pts',(20.757030176897,14.1208391087228,-3.82682916955609));
#37884=CARTESIAN_POINT('Ctrl Pts',(20.7519216253324,14.1886524290741,-3.91212743179073));
#37885=CARTESIAN_POINT('Ctrl Pts',(20.7468130737678,14.2536951325735,-3.99955619341295));
#37886=CARTESIAN_POINT('Ctrl Pts',(20.7417045222033,14.3158368081123,-4.08892028122819));
#37887=CARTESIAN_POINT('Ctrl Pts',(20.7349885913884,14.3975310395132,-4.20640231571828));
#37888=CARTESIAN_POINT('Ctrl Pts',(20.7282726605735,14.4743500912044,-4.3274317992558));
#37889=CARTESIAN_POINT('Ctrl Pts',(20.7215567297586,14.5459825288401,-4.45157243139028));
#37890=CARTESIAN_POINT('Ctrl Pts',(20.7148461574089,14.6175578128304,-4.57561401496664));
#37891=CARTESIAN_POINT('Ctrl Pts',(20.7081355850593,14.6839545411525,-4.70276148394193));
#37892=CARTESIAN_POINT('Ctrl Pts',(20.7014250127097,14.7449047642867,-4.83254991711475));
#37893=CARTESIAN_POINT('Ctrl Pts',(20.6947184269592,14.8058187782729,-4.962261245917));
#37894=CARTESIAN_POINT('Ctrl Pts',(20.6880118412087,14.8612925759747,-5.09461007959434));
#37895=CARTESIAN_POINT('Ctrl Pts',(20.6813052554582,14.9111043584523,-5.22910735524996));
#37896=CARTESIAN_POINT('Ctrl Pts',(20.6746012879102,14.9608966947709,-5.36355212414347));
#37897=CARTESIAN_POINT('Ctrl Pts',(20.6678973203622,15.0050312919063,-5.50014331759118));
#37898=CARTESIAN_POINT('Ctrl Pts',(20.6611933528142,15.0433346977241,-5.63837245788636));
#37899=CARTESIAN_POINT('Ctrl Pts',(20.6544893167563,15.0816384949762,-5.77660301078764));
#37900=CARTESIAN_POINT('Ctrl Pts',(20.6477852806984,15.1141108743886,-5.91647119019885));
#37901=CARTESIAN_POINT('Ctrl Pts',(20.6410812446405,15.1406283667068,-6.05745371870328));
#37902=CARTESIAN_POINT('Ctrl Pts',(20.6343768576303,15.1671472471998,-6.19844362755812));
#37903=CARTESIAN_POINT('Ctrl Pts',(20.6276724706202,15.1877105506822,-6.34054763828436));
#37904=CARTESIAN_POINT('Ctrl Pts',(20.62096808361,15.2022460867859,-6.48323299350801));
#37905=CARTESIAN_POINT('Ctrl Pts',(20.6142621064915,15.2167850703453,-6.62595219003299));
#37906=CARTESIAN_POINT('Ctrl Pts',(20.6075561293729,15.2252934010757,-6.76925263776888));
#37907=CARTESIAN_POINT('Ctrl Pts',(20.6008501522544,15.227750853798,-6.91259730125182));
#37908=CARTESIAN_POINT('Ctrl Pts',(20.5941413450238,15.2302093436348,-7.05600246023726));
#37909=CARTESIAN_POINT('Ctrl Pts',(20.5874325377932,15.2266118621726,-7.19945150257357));
#37910=CARTESIAN_POINT('Ctrl Pts',(20.5807237305627,15.2169902963606,-7.34240835917999));
#37911=CARTESIAN_POINT('Ctrl Pts',(20.5740069743706,15.2073573303917,-7.48553459888302));
#37912=CARTESIAN_POINT('Ctrl Pts',(20.5672902181786,15.1916860472491,-7.62816711857751));
#37913=CARTESIAN_POINT('Ctrl Pts',(20.5605734619866,15.1700602117555,-7.76977513058491));
#37914=CARTESIAN_POINT('Ctrl Pts',(20.5538523224127,15.1484202631557,-7.9114755565444));
#37915=CARTESIAN_POINT('Ctrl Pts',(20.5471311828389,15.1208180850618,-8.05214977921533));
#37916=CARTESIAN_POINT('Ctrl Pts',(20.5404100432651,15.0873882866751,-8.19127861428367));
#37917=CARTESIAN_POINT('Ctrl Pts',(20.5336789815349,15.0539091371805,-8.33061283982664));
#37918=CARTESIAN_POINT('Ctrl Pts',(20.5269479198048,15.0145852798129,-8.46839676418098));
#37919=CARTESIAN_POINT('Ctrl Pts',(20.5202168580746,14.9696010262843,-8.60412688256326));
#37920=CARTESIAN_POINT('Ctrl Pts',(20.5164823161787,14.9446427676626,-8.67943295372376));
#37921=CARTESIAN_POINT('Ctrl Pts',(20.5127477742828,14.9179429442996,-8.75410715651371));
#37922=CARTESIAN_POINT('Ctrl Pts',(20.5090132323869,14.8895392850499,-8.82806646618269));
#37923=CARTESIAN_POINT('Ctrl Pts',(20.5025200449742,14.8401543034763,-8.95665831813692));
#37924=CARTESIAN_POINT('Ctrl Pts',(20.4960268575615,14.7854588635406,-9.08349642489812));
#37925=CARTESIAN_POINT('Ctrl Pts',(20.4895336701487,14.7255962343738,-9.20809882124304));
#37926=CARTESIAN_POINT('Ctrl Pts',(20.4830489427434,14.6658116005356,-9.33253887248255));
#37927=CARTESIAN_POINT('Ctrl Pts',(20.4765642153381,14.6008733355466,-9.45474864825517));
#37928=CARTESIAN_POINT('Ctrl Pts',(20.4700794879328,14.5309741013637,-9.57426236716936));
#37929=CARTESIAN_POINT('Ctrl Pts',(20.4636015680842,14.46114824621,-9.69365062261074));
#37930=CARTESIAN_POINT('Ctrl Pts',(20.4571236482356,14.3863719800204,-9.81034810648507));
#37931=CARTESIAN_POINT('Ctrl Pts',(20.450645728387,14.3068853679125,-9.92391047878529));
#37932=CARTESIAN_POINT('Ctrl Pts',(20.4441729717852,14.227462110864,-10.0373823358321));
#37933=CARTESIAN_POINT('Ctrl Pts',(20.4377002151834,14.1433362049446,-10.1477237249245));
#37934=CARTESIAN_POINT('Ctrl Pts',(20.4312274585816,14.0547925601806,-10.2545167562928));
#37935=CARTESIAN_POINT('Ctrl Pts',(20.4247576155,13.9662887707232,-10.3612617179322));
#37936=CARTESIAN_POINT('Ctrl Pts',(20.4182877724184,13.8733714499816,-10.464461188119));
#37937=CARTESIAN_POINT('Ctrl Pts',(20.4118179293369,13.7763673517941,-10.5637283171446));
#37938=CARTESIAN_POINT('Ctrl Pts',(20.4053495189975,13.679384735096,-10.6629734635342));
#37939=CARTESIAN_POINT('Ctrl Pts',(20.3988811086581,13.5783174199717,-10.758287712789));
#37940=CARTESIAN_POINT('Ctrl Pts',(20.3924126983188,13.4735304075049,-10.8493196325692));
#37941=CARTESIAN_POINT('Ctrl Pts',(20.385944242306,13.3687426551373,-10.9403521951256));
#37942=CARTESIAN_POINT('Ctrl Pts',(20.3794757862932,13.2602354559434,-11.0271021046895));
#37943=CARTESIAN_POINT('Ctrl Pts',(20.3730073302804,13.1484079939686,-11.1092572959055));
#37944=CARTESIAN_POINT('Ctrl Pts',(20.3665373502499,13.0365541845895,-11.1914318435122));
#37945=CARTESIAN_POINT('Ctrl Pts',(20.3600673702195,12.9213788801603,-11.2690092826117));
#37946=CARTESIAN_POINT('Ctrl Pts',(20.353597390189,12.8033109676334,-11.3417203859027));
#37947=CARTESIAN_POINT('Ctrl Pts',(20.3471201497813,12.6851105635712,-11.4145130829604));
#37948=CARTESIAN_POINT('Ctrl Pts',(20.3406429093736,12.5640114110033,-11.4824283276885));
#37949=CARTESIAN_POINT('Ctrl Pts',(20.3341656689659,12.4404681640428,-11.5452422536957));
#37950=CARTESIAN_POINT('Ctrl Pts',(20.3276847808162,12.3168553420999,-11.6080915541802));
#37951=CARTESIAN_POINT('Ctrl Pts',(20.3212038926665,12.1907960499717,-11.6658336502188));
#37952=CARTESIAN_POINT('Ctrl Pts',(20.3147230045168,12.0627645335034,-11.7182930434107));
#37953=CARTESIAN_POINT('Ctrl Pts',(20.3082311045841,11.9345154765905,-11.770841571216));
#37954=CARTESIAN_POINT('Ctrl Pts',(20.3017392046513,11.8042878781064,-11.8180893292629));
#37955=CARTESIAN_POINT('Ctrl Pts',(20.2952473047185,11.6725715143819,-11.8599106269049));
#37956=CARTESIAN_POINT('Ctrl Pts',(20.2889388506692,11.5445771465229,-11.9005501526507));
#37957=CARTESIAN_POINT('Ctrl Pts',(20.2826303966198,11.4151773566558,-11.9360657571026));
#37958=CARTESIAN_POINT('Ctrl Pts',(20.2763219425705,11.2848280760658,-11.9663888326081));
#37959=CARTESIAN_POINT('Ctrl Pts',(20.2664266823321,11.0803659299939,-12.0139527398677));
#37960=CARTESIAN_POINT('Ctrl Pts',(20.2565314220938,10.8730095382161,-12.0488763230015));
#37961=CARTESIAN_POINT('Ctrl Pts',(20.2466361618554,10.6640303707002,-12.0709050753094));
#37962=CARTESIAN_POINT('Ctrl Pts',(20.2383086093597,10.4881598078176,-12.0894438086868));
#37963=CARTESIAN_POINT('Ctrl Pts',(20.2299810568641,10.3111395726563,-12.098850629708));
#37964=CARTESIAN_POINT('Ctrl Pts',(20.2216535043684,10.1337426824875,-12.0989982349129));
#37965=CARTESIAN_POINT('Origin',(26.8463464956315,10.1295,-7.));
#37966=CARTESIAN_POINT('',(22.6904763725673,6.08319878352126,-3.8972193977784));
#37967=CARTESIAN_POINT('',(22.5651720735025,6.0835080422226,-3.89745662547144));
#37968=CARTESIAN_POINT('',(26.8463464956315,6.08319878352126,-3.89721939777839));
#37969=CARTESIAN_POINT('',(23.2216535038443,10.1293865183057,-12.0989488216269));
#37970=CARTESIAN_POINT('Ctrl Pts',(23.2216535036445,10.1293865128977,-12.0989999987371));
#37971=CARTESIAN_POINT('Ctrl Pts',(23.2144616473686,9.97576251488196,-12.0989965795681));
#37972=CARTESIAN_POINT('Ctrl Pts',(23.2072697910928,9.82216920243597,-12.0920461851236));
#37973=CARTESIAN_POINT('Ctrl Pts',(23.2000779348169,9.66922023943467,-12.0781830945737));
#37974=CARTESIAN_POINT('Ctrl Pts',(23.1950396449697,9.56207110048146,-12.0684712391514));
#37975=CARTESIAN_POINT('Ctrl Pts',(23.1900013551225,9.45523816700231,-12.0553678804514));
#37976=CARTESIAN_POINT('Ctrl Pts',(23.1849630652753,9.34893090479854,-12.0388999680105));
#37977=CARTESIAN_POINT('Ctrl Pts',(23.1780322106042,9.20269077031505,-12.0162461089975));
#37978=CARTESIAN_POINT('Ctrl Pts',(23.1711013559331,9.05741147522505,-11.9872176032497));
#37979=CARTESIAN_POINT('Ctrl Pts',(23.1641705012619,8.91365350675345,-11.9519206682721));
#37980=CARTESIAN_POINT('Ctrl Pts',(23.1572409972287,8.76992355285804,-11.9166306117213));
#37981=CARTESIAN_POINT('Ctrl Pts',(23.1503114931954,8.6277146554914,-11.8750746419589));
#37982=CARTESIAN_POINT('Ctrl Pts',(23.1433819891621,8.48757530416641,-11.8274096877323));
#37983=CARTESIAN_POINT('Ctrl Pts',(23.1364522650283,8.34743150162177,-11.7797432195329));
#37984=CARTESIAN_POINT('Ctrl Pts',(23.1295225408946,8.20935769125029,-11.7259674819089));
#37985=CARTESIAN_POINT('Ctrl Pts',(23.1225928167608,8.07388595843718,-11.6662888800555));
#37986=CARTESIAN_POINT('Ctrl Pts',(23.1156634748197,7.93842169724982,-11.6066135696355));
#37987=CARTESIAN_POINT('Ctrl Pts',(23.1087341328786,7.80555952912581,-11.5410361807239));
#37988=CARTESIAN_POINT('Ctrl Pts',(23.1018047909375,7.67581036564082,-11.4698107541862));
#37989=CARTESIAN_POINT('Ctrl Pts',(23.0948738940547,7.54603208649339,-11.3985693446901));
#37990=CARTESIAN_POINT('Ctrl Pts',(23.0879429971719,7.4193684981623,-11.321677524493));
#37991=CARTESIAN_POINT('Ctrl Pts',(23.0810121002891,7.29630531956496,-11.2394349744694));
#37992=CARTESIAN_POINT('Ctrl Pts',(23.0768805403151,7.22294642942954,-11.1904095693044));
#37993=CARTESIAN_POINT('Ctrl Pts',(23.0727489803412,7.15086641510118,-11.139483671144));
#37994=CARTESIAN_POINT('Ctrl Pts',(23.0686174203672,7.08016321996373,-11.0867280557823));
#37995=CARTESIAN_POINT('Ctrl Pts',(23.0616832524995,6.96149912529913,-10.9981861260548));
#37996=CARTESIAN_POINT('Ctrl Pts',(23.0547490846318,6.84667369731443,-10.9044571565873));
#37997=CARTESIAN_POINT('Ctrl Pts',(23.0478149167641,6.73613270977454,-10.805897979929));
#37998=CARTESIAN_POINT('Ctrl Pts',(23.0408820598754,6.62561262119616,-10.7073574369422));
#37999=CARTESIAN_POINT('Ctrl Pts',(23.0339492029866,6.51937560346518,-10.603988728551));
#38000=CARTESIAN_POINT('Ctrl Pts',(23.0270163460979,6.4178330651246,-10.4961878617364));
#38001=CARTESIAN_POINT('Ctrl Pts',(23.0200832422255,6.3162869093225,-10.3883831545067));
#38002=CARTESIAN_POINT('Ctrl Pts',(23.0131501383532,6.21943579656273,-10.2761462111623));
#38003=CARTESIAN_POINT('Ctrl Pts',(23.0062170344808,6.127653461249,-10.159909062028));
#38004=CARTESIAN_POINT('Ctrl Pts',(22.9992843056565,6.0358760909238,-10.0436782007715));
#38005=CARTESIAN_POINT('Ctrl Pts',(22.9923515768321,5.94916715343914,-9.92344782666485));
#38006=CARTESIAN_POINT('Ctrl Pts',(22.9854188480078,5.86785936094203,-9.79968213615932));
#38007=CARTESIAN_POINT('Ctrl Pts',(22.9784845828,5.78653354957469,-9.67588901755805));
#38008=CARTESIAN_POINT('Ctrl Pts',(22.9715503175923,5.71061145639965,-9.54855929336527));
#38009=CARTESIAN_POINT('Ctrl Pts',(22.9646160523846,5.64038215784226,-9.41818568336285));
#38010=CARTESIAN_POINT('Ctrl Pts',(22.9605012934094,5.59870843641641,-9.34082262241638));
#38011=CARTESIAN_POINT('Ctrl Pts',(22.9563865344342,5.55903840082034,-9.26238827233416));
#38012=CARTESIAN_POINT('Ctrl Pts',(22.952271775459,5.52142478724157,-9.18298965493686));
#38013=CARTESIAN_POINT('Ctrl Pts',(22.9453381235802,5.45804326136591,-9.04919752373096));
#38014=CARTESIAN_POINT('Ctrl Pts',(22.9384044717014,5.40048158569252,-8.91262014426123));
#38015=CARTESIAN_POINT('Ctrl Pts',(22.9314708198227,5.34896652564976,-8.77378146923933));
#38016=CARTESIAN_POINT('Ctrl Pts',(22.9245384819542,5.29746122832944,-8.63496910581344));
#38017=CARTESIAN_POINT('Ctrl Pts',(22.9176061440857,5.25200037531062,-8.49389661159093));
#38018=CARTESIAN_POINT('Ctrl Pts',(22.9106738062172,5.21276202370896,-8.3511064623106));
#38019=CARTESIAN_POINT('Ctrl Pts',(22.9037412208191,5.17352227104248,-8.20831121449157));
#38020=CARTESIAN_POINT('Ctrl Pts',(22.896808635421,5.14050555518979,-8.06379850674376));
#38021=CARTESIAN_POINT('Ctrl Pts',(22.8898760500228,5.1138397764683,-7.9181250035164));
#38022=CARTESIAN_POINT('Ctrl Pts',(22.8829438381066,5.08717543432276,-7.77245934821475));
#38023=CARTESIAN_POINT('Ctrl Pts',(22.8760116261904,5.06686140326674,-7.62563334790481));
#38024=CARTESIAN_POINT('Ctrl Pts',(22.8690794142742,5.05297427438577,-7.4782128785143));
#38025=CARTESIAN_POINT('Ctrl Pts',(22.8621456590075,5.03908405374907,-7.33075958822291));
#38026=CARTESIAN_POINT('Ctrl Pts',(22.8552119037409,5.03162362532709,-7.18271189362287));
#38027=CARTESIAN_POINT('Ctrl Pts',(22.8482781484743,5.03061766757055,-7.03464043935698));
#38028=CARTESIAN_POINT('Ctrl Pts',(22.8441608091664,5.03002031891117,-6.94671399898356));
#38029=CARTESIAN_POINT('Ctrl Pts',(22.8400434698586,5.03169789774968,-6.85877924044733));
#38030=CARTESIAN_POINT('Ctrl Pts',(22.8359261305508,5.03564687217782,-6.77095565456406));
#38031=CARTESIAN_POINT('Ctrl Pts',(22.8289927902407,5.04229669662495,-6.62306626225001));
#38032=CARTESIAN_POINT('Ctrl Pts',(22.8220594499305,5.05539250041431,-6.47544107236297));
#38033=CARTESIAN_POINT('Ctrl Pts',(22.8151261096204,5.07488932497261,-6.32864917971362));
#38034=CARTESIAN_POINT('Ctrl Pts',(22.8081940896352,5.09438243672549,-6.18188524083354));
#38035=CARTESIAN_POINT('Ctrl Pts',(22.80126206965,5.12027409374892,-6.03595461015682));
#38036=CARTESIAN_POINT('Ctrl Pts',(22.7943300496648,5.15246762548965,-5.8914199428657));
#38037=CARTESIAN_POINT('Ctrl Pts',(22.7873977885485,5.18466227708635,-5.74688024791841));
#38038=CARTESIAN_POINT('Ctrl Pts',(22.7804655274321,5.22315917345076,-5.60373693696194));
#38039=CARTESIAN_POINT('Ctrl Pts',(22.7735332663157,5.26781068180791,-5.46254171654092));
#38040=CARTESIAN_POINT('Ctrl Pts',(22.7666013815341,5.312459766149,-5.3213541612469));
#38041=CARTESIAN_POINT('Ctrl Pts',(22.7596694967524,5.36326269333952,-5.18211479983463));
#38042=CARTESIAN_POINT('Ctrl Pts',(22.7527376119708,5.42002218067546,-5.04535945266396));
#38043=CARTESIAN_POINT('Ctrl Pts',(22.745804185402,5.47679429243441,-4.90857368842235));
#38044=CARTESIAN_POINT('Ctrl Pts',(22.7388707588332,5.53952548479134,-4.77427334785542));
#38045=CARTESIAN_POINT('Ctrl Pts',(22.7319373322645,5.60797037248123,-4.6429741563848));
#38046=CARTESIAN_POINT('Ctrl Pts',(22.7278183833905,5.6486315073879,-4.56497309132771));
#38047=CARTESIAN_POINT('Ctrl Pts',(22.7236994345166,5.69130821780808,-4.48803078158948));
#38048=CARTESIAN_POINT('Ctrl Pts',(22.7195804856426,5.73594135530312,-4.41225128043519));
#38049=CARTESIAN_POINT('Ctrl Pts',(22.7126467717647,5.811075428178,-4.28468636159476));
#38050=CARTESIAN_POINT('Ctrl Pts',(22.7057130578868,5.89178185883559,-4.16037391185343));
#38051=CARTESIAN_POINT('Ctrl Pts',(22.6987793440089,5.97775436558227,-4.03979575247022));
#38052=CARTESIAN_POINT('Ctrl Pts',(22.6960116868617,6.01207110073318,-3.99166584539737));
#38053=CARTESIAN_POINT('Ctrl Pts',(22.6932440297145,6.04722637638245,-3.944130608536));
#38054=CARTESIAN_POINT('Ctrl Pts',(22.6904763725673,6.08319878352126,-3.8972193977784));
#38055=CARTESIAN_POINT('',(23.534,15.0539061944433,-8.32288496556904));
#38056=CARTESIAN_POINT('Ctrl Pts',(23.534,15.0539061944433,-8.32288496556903));
#38057=CARTESIAN_POINT('Ctrl Pts',(23.4952181183639,14.8390046351781,-9.12285064450927));
#38058=CARTESIAN_POINT('Ctrl Pts',(23.4176543550918,14.012227531697,-10.6153576611852));
#38059=CARTESIAN_POINT('Ctrl Pts',(23.3135388565479,12.092423032665,-11.8658595382605));
#38060=CARTESIAN_POINT('Ctrl Pts',(23.2482052396401,10.6965329474454,-12.0983697707759));
#38061=CARTESIAN_POINT('Ctrl Pts',(23.2216535043684,10.1293865324873,-12.0988146186003));
#38062=CARTESIAN_POINT('',(23.5339999999999,15.0538811994916,-5.6770219948566));
#38063=CARTESIAN_POINT('Origin',(23.534,10.1295,-7.));
#38064=CARTESIAN_POINT('',(23.0963464956316,10.1294332241516,-12.0990513781753));
#38065=CARTESIAN_POINT('Ctrl Pts',(23.5339999999999,15.0538811994916,-5.6770219948566));
#38066=CARTESIAN_POINT('Ctrl Pts',(23.5270930717027,15.0921506970965,-5.8194685009863));
#38067=CARTESIAN_POINT('Ctrl Pts',(23.5201861434054,15.1242415793792,-5.96360031998381));
#38068=CARTESIAN_POINT('Ctrl Pts',(23.5132792151082,15.1500258622284,-6.10886529262073));
#38069=CARTESIAN_POINT('Ctrl Pts',(23.5063724323829,15.1758096016423,-6.25412720362094));
#38070=CARTESIAN_POINT('Ctrl Pts',(23.4994656496576,15.1952869431655,-6.40052189108961));
#38071=CARTESIAN_POINT('Ctrl Pts',(23.4925588669324,15.2083811232991,-6.54748753012045));
#38072=CARTESIAN_POINT('Ctrl Pts',(23.4856526906085,15.2214741537902,-6.69444026586755));
#38073=CARTESIAN_POINT('Ctrl Pts',(23.4787465142847,15.2281851137662,-6.84196351862882));
#38074=CARTESIAN_POINT('Ctrl Pts',(23.4718403379609,15.2284891702847,-6.98949089349636));
#38075=CARTESIAN_POINT('Ctrl Pts',(23.4649324938645,15.2287933002297,-7.13705389474971));
#38076=CARTESIAN_POINT('Ctrl Pts',(23.4580246497681,15.2226874332482,-7.28462068429066));
#38077=CARTESIAN_POINT('Ctrl Pts',(23.4511168056718,15.2101988752891,-7.43162476601365));
#38078=CARTESIAN_POINT('Ctrl Pts',(23.4457234039484,15.2004482484538,-7.54640038292906));
#38079=CARTESIAN_POINT('Ctrl Pts',(23.4403300022249,15.186807817628,-7.66083293227476));
#38080=CARTESIAN_POINT('Ctrl Pts',(23.4349366005015,15.1693125726679,-7.77465491180164));
#38081=CARTESIAN_POINT('Ctrl Pts',(23.4280029490964,15.1468210291077,-7.92098221481945));
#38082=CARTESIAN_POINT('Ctrl Pts',(23.4210692976913,15.1179485596679,-8.06635451124193));
#38083=CARTESIAN_POINT('Ctrl Pts',(23.4141356462862,15.0828010075303,-8.21021077866611));
#38084=CARTESIAN_POINT('Ctrl Pts',(23.4072033088961,15.0476601163007,-8.35403978349831));
#38085=CARTESIAN_POINT('Ctrl Pts',(23.4002709715061,15.0062465934393,-8.49635301161162));
#38086=CARTESIAN_POINT('Ctrl Pts',(23.3933386341161,14.958717003046,-8.63660139847525));
#38087=CARTESIAN_POINT('Ctrl Pts',(23.3864060491991,14.9111857155543,-8.77685479306806));
#38088=CARTESIAN_POINT('Ctrl Pts',(23.379473464282,14.857538026485,-8.91504288474696));
#38089=CARTESIAN_POINT('Ctrl Pts',(23.372540879365,14.79797999132,-9.05063296829173));
#38090=CARTESIAN_POINT('Ctrl Pts',(23.3656086679301,14.7384251647511,-9.18621574713243));
#38091=CARTESIAN_POINT('Ctrl Pts',(23.3586764564952,14.6729607630339,-9.31920049562694));
#38092=CARTESIAN_POINT('Ctrl Pts',(23.3517442450604,14.6018404979881,-9.44907563583814));
#38093=CARTESIAN_POINT('Ctrl Pts',(23.3448104902714,14.530704399069,-9.57897969082492));
#38094=CARTESIAN_POINT('Ctrl Pts',(23.3378767354823,14.453910079615,-9.70577246416573));
#38095=CARTESIAN_POINT('Ctrl Pts',(23.3309429806933,14.3717569175791,-9.82896752283444));
#38096=CARTESIAN_POINT('Ctrl Pts',(23.3268256389933,14.3229734445361,-9.90212213642044));
#38097=CARTESIAN_POINT('Ctrl Pts',(23.3227082972933,14.2723012354768,-9.97400865986319));
#38098=CARTESIAN_POINT('Ctrl Pts',(23.3185909555933,14.2198101839654,-10.0445301113552));
#38099=CARTESIAN_POINT('Ctrl Pts',(23.3116576153536,14.1314186084821,-10.1632837278912));
#38100=CARTESIAN_POINT('Ctrl Pts',(23.304724275114,14.0378366099381,-10.2782059009288));
#38101=CARTESIAN_POINT('Ctrl Pts',(23.2977909348743,13.9394203703912,-10.3888505088419));
#38102=CARTESIAN_POINT('Ctrl Pts',(23.2908589149614,13.8410228724023,-10.4994740465298));
#38103=CARTESIAN_POINT('Ctrl Pts',(23.2839268950485,13.7377931897414,-10.6058213974011));
#38104=CARTESIAN_POINT('Ctrl Pts',(23.2769948751356,13.6301267227303,-10.7074807549205));
#38105=CARTESIAN_POINT('Ctrl Pts',(23.2700626140937,13.5224565105608,-10.8091436486423));
#38106=CARTESIAN_POINT('Ctrl Pts',(23.2631303530518,13.410349443299,-10.9061179932801));
#38107=CARTESIAN_POINT('Ctrl Pts',(23.2561980920098,13.2942369915247,-10.9980296115056));
#38108=CARTESIAN_POINT('Ctrl Pts',(23.2492662073036,13.1781308432153,-11.089936240071));
#38109=CARTESIAN_POINT('Ctrl Pts',(23.2423343225974,13.0580200053115,-11.1767804876996));
#38110=CARTESIAN_POINT('Ctrl Pts',(23.2354024378912,12.9343681645872,-11.2582291600248));
#38111=CARTESIAN_POINT('Ctrl Pts',(23.2284690113988,12.8106888212852,-11.339695948121));
#38112=CARTESIAN_POINT('Ctrl Pts',(23.2215355849065,12.6834671776638,-11.4157645810553));
#38113=CARTESIAN_POINT('Ctrl Pts',(23.2146021584141,12.5531954963905,-11.4861454658511));
#38114=CARTESIAN_POINT('Ctrl Pts',(23.2104832091711,12.4758048377378,-11.5279567250417));
#38115=CARTESIAN_POINT('Ctrl Pts',(23.2063642599281,12.3973382765711,-11.5677615089315));
#38116=CARTESIAN_POINT('Ctrl Pts',(23.2022453106851,12.3179031154636,-11.6055067912478));
#38117=CARTESIAN_POINT('Ctrl Pts',(23.1953326016546,12.1845894660025,-11.6688535669748));
#38118=CARTESIAN_POINT('Ctrl Pts',(23.1884198926241,12.0484976489229,-11.7264202163307));
#38119=CARTESIAN_POINT('Ctrl Pts',(23.1815071835936,11.9101480240635,-11.7779800768106));
#38120=CARTESIAN_POINT('Ctrl Pts',(23.1744104595967,11.7681155591704,-11.8309124507215));
#38121=CARTESIAN_POINT('Ctrl Pts',(23.1673137355999,11.6237037330732,-11.8775136140333));
#38122=CARTESIAN_POINT('Ctrl Pts',(23.1602170116031,11.4774963192628,-11.9175915775158));
#38123=CARTESIAN_POINT('Ctrl Pts',(23.1533056473611,11.3351077055635,-11.9566227422935));
#38124=CARTESIAN_POINT('Ctrl Pts',(23.1463942831192,11.1910164761425,-11.9894671487316));
#38125=CARTESIAN_POINT('Ctrl Pts',(23.1394829188772,11.045776141037,-12.0159983087484));
#38126=CARTESIAN_POINT('Ctrl Pts',(23.132293515003,10.8946928828906,-12.0435967998619));
#38127=CARTESIAN_POINT('Ctrl Pts',(23.1251041111287,10.7423665149036,-12.0643634254656));
#38128=CARTESIAN_POINT('Ctrl Pts',(23.1179147072544,10.5894305429874,-12.0782147350843));
#38129=CARTESIAN_POINT('Ctrl Pts',(23.1107253033801,10.4364945710712,-12.092066044703));
#38130=CARTESIAN_POINT('Ctrl Pts',(23.1035358995059,10.2829494015725,-12.0990020099706));
#38131=CARTESIAN_POINT('Ctrl Pts',(23.0963464956316,10.1294332248244,-12.0989999995628));
#38132=CARTESIAN_POINT('Ctrl Pts',(23.0963464956316,10.1294332206623,-12.0993178216526));
#38133=CARTESIAN_POINT('Ctrl Pts',(23.0928642190134,10.0550711278111,-12.0993673700521));
#38134=CARTESIAN_POINT('Ctrl Pts',(23.0506000607591,9.15256913101046,-12.0800148503643));
#38135=CARTESIAN_POINT('Ctrl Pts',(22.9695540208687,7.44243506000627,-11.5744658280441));
#38136=CARTESIAN_POINT('Ctrl Pts',(22.8532083759605,5.61311993670382,-9.783588785421));
#38137=CARTESIAN_POINT('Ctrl Pts',(22.7368627310523,4.83541687908909,-7.34457045164505));
#38138=CARTESIAN_POINT('Ctrl Pts',(22.640850630233,5.21088719501814,-5.26560593676018));
#38139=CARTESIAN_POINT('Ctrl Pts',(22.5836204110498,5.84364847870133,-4.21017314688403));
#38140=CARTESIAN_POINT('Ctrl Pts',(22.5651720735026,6.08350804222181,-3.89745662547247));
#38141=CARTESIAN_POINT('Origin',(-18.734,19.211,1.76670989022852));
#38142=CARTESIAN_POINT('',(-17.1724222554293,21.243756036567,-21.2501821897702));
#38143=CARTESIAN_POINT('',(-17.176309351333,21.2386979557192,-21.3166133841489));
#38144=CARTESIAN_POINT('',(-17.1744642439897,21.2411350264762,1.76670989022852));
#38145=CARTESIAN_POINT('',(-21.2914665292272,19.2141433713253,-21.8332901097715));
#38146=CARTESIAN_POINT('Ctrl Pts',(-17.1763093513331,21.2386979557192,-21.3166133841489));
#38147=CARTESIAN_POINT('Ctrl Pts',(-16.9218454614608,21.0458242180231,-21.3324492449635));
#38148=CARTESIAN_POINT('Ctrl Pts',(-16.1161223190266,20.1710072681535,-21.3906770413387));
#38149=CARTESIAN_POINT('Ctrl Pts',(-16.015951705204,17.8786575813002,-21.4912967732743));
#38150=CARTESIAN_POINT('Ctrl Pts',(-18.3819424961549,16.2052786378474,-21.6184725799557));
#38151=CARTESIAN_POINT('Ctrl Pts',(-20.7940989859098,17.1742606647151,-21.7324703587881));
#38152=CARTESIAN_POINT('Ctrl Pts',(-21.2869488363774,18.6256784793645,-21.80407620206));
#38153=CARTESIAN_POINT('Ctrl Pts',(-21.2914665292272,19.2141433713253,-21.8332901097715));
#38154=CARTESIAN_POINT('',(-19.3957372685686,21.6839949024184,-22.));
#38155=CARTESIAN_POINT('Ctrl Pts',(-21.2914665292272,19.2141433713253,-21.8332901097715));
#38156=CARTESIAN_POINT('Ctrl Pts',(-21.2935044038853,19.4795925132556,-21.8464681376205));
#38157=CARTESIAN_POINT('Ctrl Pts',(-21.1334432779756,20.5957914633395,-21.90203810103));
#38158=CARTESIAN_POINT('Ctrl Pts',(-20.2191097516038,21.4636724677035,-21.9576080644395));
#38159=CARTESIAN_POINT('Ctrl Pts',(-19.3957372685686,21.6839949024184,-22.));
#38160=CARTESIAN_POINT('',(-18.0722321029123,21.6839867064714,-21.999999999982));
#38161=CARTESIAN_POINT('Origin',(-18.734,19.211,-22.));
#38162=CARTESIAN_POINT('',(-21.2939992552807,19.2090473192565,-21.7667098902285));
#38163=CARTESIAN_POINT('Ctrl Pts',(-21.2939992552807,19.2090473192565,-21.7667098902285));
#38164=CARTESIAN_POINT('Ctrl Pts',(-21.2940622859128,19.291681601191,-21.7708336286224));
#38165=CARTESIAN_POINT('Ctrl Pts',(-21.2901200772654,19.3744638362772,-21.7749573670163));
#38166=CARTESIAN_POINT('Ctrl Pts',(-21.2821561956048,19.456967483218,-21.7790811054102));
#38167=CARTESIAN_POINT('Ctrl Pts',(-21.2742021181198,19.5393695615683,-21.7831997671522));
#38168=CARTESIAN_POINT('Ctrl Pts',(-21.2622362475653,19.621493264571,-21.7873184288942));
#38169=CARTESIAN_POINT('Ctrl Pts',(-21.2462941860021,19.7029125155758,-21.7914370906363));
#38170=CARTESIAN_POINT('Ctrl Pts',(-21.2303628161442,19.7842771619339,-21.795552990156));
#38171=CARTESIAN_POINT('Ctrl Pts',(-21.2104606359213,19.8649378301924,-21.7996688896757));
#38172=CARTESIAN_POINT('Ctrl Pts',(-21.1866748718834,19.9444752707705,-21.8037847891954));
#38173=CARTESIAN_POINT('Ctrl Pts',(-21.1628974693084,20.0239847513738,-21.8078992418438));
#38174=CARTESIAN_POINT('Ctrl Pts',(-21.1352393281534,20.102371334612,-21.8120136944921));
#38175=CARTESIAN_POINT('Ctrl Pts',(-21.1038380300699,20.1792291625614,-21.8161281471405));
#38176=CARTESIAN_POINT('Ctrl Pts',(-21.0724377503042,20.2560844980759,-21.8202424663606));
#38177=CARTESIAN_POINT('Ctrl Pts',(-21.0372947356062,20.3314107390252,-21.8243567855807));
#38178=CARTESIAN_POINT('Ctrl Pts',(-20.9985947990105,20.404821760689,-21.8284711048008));
#38179=CARTESIAN_POINT('Ctrl Pts',(-20.959859212032,20.4783004085882,-21.8325892141319));
#38180=CARTESIAN_POINT('Ctrl Pts',(-20.9175603821396,20.5498598946646,-21.836707323463));
#38181=CARTESIAN_POINT('Ctrl Pts',(-20.8719298670911,20.6191391562625,-21.8408254327941));
#38182=CARTESIAN_POINT('Ctrl Pts',(-20.8262774610213,20.6884516542547,-21.8449455177684));
#38183=CARTESIAN_POINT('Ctrl Pts',(-20.7772904689067,20.7554813685366,-21.8490656027427));
#38184=CARTESIAN_POINT('Ctrl Pts',(-20.7252420320998,20.8198987443587,-21.8531856877171));
#38185=CARTESIAN_POINT('Ctrl Pts',(-20.6731075655348,20.884422594296,-21.8573125826926));
#38186=CARTESIAN_POINT('Ctrl Pts',(-20.617901867132,20.9463251318754,-21.861439477668));
#38187=CARTESIAN_POINT('Ctrl Pts',(-20.5599360229587,21.0053125814812,-21.8655663726435));
#38188=CARTESIAN_POINT('Ctrl Pts',(-20.5193323219955,21.0466318928538,-21.8684571648312));
#38189=CARTESIAN_POINT('Ctrl Pts',(-20.477375083183,21.0865216493047,-21.871347957019));
#38190=CARTESIAN_POINT('Ctrl Pts',(-20.4341804477789,21.1248930077176,-21.8742387492067));
#38191=CARTESIAN_POINT('Ctrl Pts',(-20.3717054008517,21.1803918536987,-21.8784198790135));
#38192=CARTESIAN_POINT('Ctrl Pts',(-20.3063945881463,21.2329309746761,-21.8826010088204));
#38193=CARTESIAN_POINT('Ctrl Pts',(-20.2385603336045,21.2822069434375,-21.8867821386272));
#38194=CARTESIAN_POINT('Ctrl Pts',(-20.1708211017769,21.3314138860656,-21.8909574114772));
#38195=CARTESIAN_POINT('Ctrl Pts',(-20.1005658190123,21.3773664872955,-21.8951326843272));
#38196=CARTESIAN_POINT('Ctrl Pts',(-20.0281414820515,21.4198000870231,-21.8993079571772));
#38197=CARTESIAN_POINT('Ctrl Pts',(-19.9553662537474,21.4624392748643,-21.9035034589607));
#38198=CARTESIAN_POINT('Ctrl Pts',(-19.8804012470982,21.5015249551222,-21.9076989607443));
#38199=CARTESIAN_POINT('Ctrl Pts',(-19.8036298896135,21.5368314425696,-21.9118944625278));
#38200=CARTESIAN_POINT('Ctrl Pts',(-19.7273621652182,21.571906313488,-21.9160624411101));
#38201=CARTESIAN_POINT('Ctrl Pts',(-19.6493121425953,21.6032512322234,-21.9202304196923));
#38202=CARTESIAN_POINT('Ctrl Pts',(-19.5698807349969,21.6306907647179,-21.9243983982746));
#38203=CARTESIAN_POINT('Ctrl Pts',(-19.4904743833841,21.6581216416371,-21.9285650621022));
#38204=CARTESIAN_POINT('Ctrl Pts',(-19.4096879474075,21.6816494286122,-21.9327317259298));
#38205=CARTESIAN_POINT('Ctrl Pts',(-19.3279406124946,21.7011474953965,-21.9368983897574));
#38206=CARTESIAN_POINT('Ctrl Pts',(-19.2461944456416,21.7206452835795,-21.941064994049));
#38207=CARTESIAN_POINT('Ctrl Pts',(-19.1634878556314,21.7361133602598,-21.9452315983405));
#38208=CARTESIAN_POINT('Ctrl Pts',(-19.0802520749481,21.7474758032739,-21.9493982026321));
#38209=CARTESIAN_POINT('Ctrl Pts',(-18.9960132117624,21.7589751761959,-21.9536150190779));
#38210=CARTESIAN_POINT('Ctrl Pts',(-18.9112327938041,21.7662692144946,-21.9578318355238));
#38211=CARTESIAN_POINT('Ctrl Pts',(-18.8263632855961,21.7693332510589,-21.9620486519696));
#38212=CARTESIAN_POINT('Ctrl Pts',(-18.742382112111,21.7723652161511,-21.9662213307204));
#38213=CARTESIAN_POINT('Ctrl Pts',(-18.6583141699189,21.7712553860981,-21.9703940094712));
#38214=CARTESIAN_POINT('Ctrl Pts',(-18.5745961490186,21.7660323701065,-21.9745666882221));
#38215=CARTESIAN_POINT('Ctrl Pts',(-18.489549801391,21.7607264822116,-21.9788055735154));
#38216=CARTESIAN_POINT('Ctrl Pts',(-18.404865068191,21.7511758035055,-21.9830444588087));
#38217=CARTESIAN_POINT('Ctrl Pts',(-18.3209906477349,21.7374645801874,-21.987283344102));
#38218=CARTESIAN_POINT('Ctrl Pts',(-18.2371162272788,21.7237533568693,-21.9915222293954));
#38219=CARTESIAN_POINT('Ctrl Pts',(-18.15405258588,21.7058817570232,-21.9957611146887));
#38220=CARTESIAN_POINT('Ctrl Pts',(-18.0722321029123,21.6839867064714,-21.999999999982));
#38221=CARTESIAN_POINT('Ctrl Pts',(-17.1724222554293,21.243756036567,-21.2501821897702));
#38222=CARTESIAN_POINT('Ctrl Pts',(-16.5648620804737,20.7701940639652,-21.2886333006738));
#38223=CARTESIAN_POINT('Ctrl Pts',(-15.7493319248272,19.1595847174514,-21.3694763471378));
#38224=CARTESIAN_POINT('Ctrl Pts',(-17.0720918435031,16.6810623606466,-21.4927113291624));
#38225=CARTESIAN_POINT('Ctrl Pts',(-19.9618263432431,16.4438210470481,-21.6198871358438));
#38226=CARTESIAN_POINT('Ctrl Pts',(-21.2281784392051,18.0973738826004,-21.7112199895325));
#38227=CARTESIAN_POINT('Ctrl Pts',(-21.2971424588611,19.0777088858588,-21.7601609076608));
#38228=CARTESIAN_POINT('Ctrl Pts',(-21.2960081347233,19.2090457869513,-21.7667098902285));
#38229=CARTESIAN_POINT('Origin',(-18.734,19.211,1.76670989022852));
#38230=CARTESIAN_POINT('',(-17.173927552048,21.2418454004354,-20.4499991710565));
#38231=CARTESIAN_POINT('',(-17.1744642439897,21.2411350264762,-20.5167504934799));
#38232=CARTESIAN_POINT('',(-17.1744642439897,21.2411350264762,1.76670989022852));
#38233=CARTESIAN_POINT('',(-21.2939288326654,19.209658289924,-21.0332900817688));
#38234=CARTESIAN_POINT('Ctrl Pts',(-17.1744642439897,21.2411350264762,-20.5167504934799));
#38235=CARTESIAN_POINT('Ctrl Pts',(-17.1078271467209,21.1899448669488,-20.5209209326673));
#38236=CARTESIAN_POINT('Ctrl Pts',(-17.0436732700516,21.1354397282691,-20.5250913718547));
#38237=CARTESIAN_POINT('Ctrl Pts',(-16.9823432210665,21.0778954252491,-20.5292618110421));
#38238=CARTESIAN_POINT('Ctrl Pts',(-16.9210263875684,21.0203635219582,-20.5334313515773));
#38239=CARTESIAN_POINT('Ctrl Pts',(-16.8625325082685,20.9597940700024,-20.5376008921125));
#38240=CARTESIAN_POINT('Ctrl Pts',(-16.8071671720215,20.8965014841359,-20.5417704326477));
#38241=CARTESIAN_POINT('Ctrl Pts',(-16.7517971586262,20.8332035514436,-20.545940325417));
#38242=CARTESIAN_POINT('Ctrl Pts',(-16.6995565149628,20.7671823751704,-20.5501102181863));
#38243=CARTESIAN_POINT('Ctrl Pts',(-16.6507112795958,20.6987863110799,-20.5542801109556));
#38244=CARTESIAN_POINT('Ctrl Pts',(-16.601814675656,20.630318317595,-20.5584543890337));
#38245=CARTESIAN_POINT('Ctrl Pts',(-16.5563208778988,20.559470824403,-20.5626286671118));
#38246=CARTESIAN_POINT('Ctrl Pts',(-16.5144529067884,20.4866216919667,-20.5668029451899));
#38247=CARTESIAN_POINT('Ctrl Pts',(-16.4725619714146,20.4137326023358,-20.5709795128277));
#38248=CARTESIAN_POINT('Ctrl Pts',(-16.434301032018,20.3388400971842,-20.5751560804656));
#38249=CARTESIAN_POINT('Ctrl Pts',(-16.3998462658687,20.2623450173186,-20.5793326481034));
#38250=CARTESIAN_POINT('Ctrl Pts',(-16.3653318783308,20.1857175684548,-20.5835164429783));
#38251=CARTESIAN_POINT('Ctrl Pts',(-16.3346369867409,20.1074824347686,-20.5877002378532));
#38252=CARTESIAN_POINT('Ctrl Pts',(-16.3078888304113,20.0280585002293,-20.5918840327281));
#38253=CARTESIAN_POINT('Ctrl Pts',(-16.2883209431143,19.9699551087057,-20.5949447306535));
#38254=CARTESIAN_POINT('Ctrl Pts',(-16.2708642318565,19.9112158548677,-20.5980054285788));
#38255=CARTESIAN_POINT('Ctrl Pts',(-16.255551151987,19.8520080403421,-20.6010661265042));
#38256=CARTESIAN_POINT('Ctrl Pts',(-16.2346154332719,19.7710603693827,-20.6052506479319));
#38257=CARTESIAN_POINT('Ctrl Pts',(-16.217610614143,19.6889352736661,-20.6094351693596));
#38258=CARTESIAN_POINT('Ctrl Pts',(-16.2046649078707,19.6060493535286,-20.6136196907873));
#38259=CARTESIAN_POINT('Ctrl Pts',(-16.1917376291181,19.5232814170601,-20.6177982557728));
#38260=CARTESIAN_POINT('Ctrl Pts',(-16.18285805684,19.4397552579917,-20.6219768207584));
#38261=CARTESIAN_POINT('Ctrl Pts',(-16.1781041141918,19.355900727772,-20.6261553857439));
#38262=CARTESIAN_POINT('Ctrl Pts',(-16.1732647974111,19.2705402879724,-20.6304089918873));
#38263=CARTESIAN_POINT('Ctrl Pts',(-16.1727008781513,19.1848400329948,-20.6346625980307));
#38264=CARTESIAN_POINT('Ctrl Pts',(-16.1764397024494,19.0992622517103,-20.6389162041741));
#38265=CARTESIAN_POINT('Ctrl Pts',(-16.180105918999,19.0153463859165,-20.6430872055358));
#38266=CARTESIAN_POINT('Ctrl Pts',(-16.1879092340601,18.9315487603075,-20.6472582068975));
#38267=CARTESIAN_POINT('Ctrl Pts',(-16.1998229072908,18.8483066546134,-20.6514292082593));
#38268=CARTESIAN_POINT('Ctrl Pts',(-16.2117325838689,18.7650924739571,-20.6555988103847));
#38269=CARTESIAN_POINT('Ctrl Pts',(-16.2277498149938,18.6824338981451,-20.6597684125102));
#38270=CARTESIAN_POINT('Ctrl Pts',(-16.2477960925062,18.6007622345654,-20.6639380146357));
#38271=CARTESIAN_POINT('Ctrl Pts',(-16.2678416593871,18.5190934662098,-20.6681074689506));
#38272=CARTESIAN_POINT('Ctrl Pts',(-16.2919158781826,18.4384119871213,-20.6722769232655));
#38273=CARTESIAN_POINT('Ctrl Pts',(-16.3198896103171,18.3591367325533,-20.6764463775805));
#38274=CARTESIAN_POINT('Ctrl Pts',(-16.3488485357306,18.2770695213161,-20.6807626738809));
#38275=CARTESIAN_POINT('Ctrl Pts',(-16.3819865976511,18.1965099318424,-20.6850789701814));
#38276=CARTESIAN_POINT('Ctrl Pts',(-16.4191057647636,18.1179013403771,-20.6893952664818));
#38277=CARTESIAN_POINT('Ctrl Pts',(-16.4550137295479,18.0418577555218,-20.6935707215798));
#38278=CARTESIAN_POINT('Ctrl Pts',(-16.4946467243009,17.9676401977747,-20.6977461766779));
#38279=CARTESIAN_POINT('Ctrl Pts',(-16.5377790112352,17.8956242481674,-20.7019216317759));
#38280=CARTESIAN_POINT('Ctrl Pts',(-16.5830936242915,17.8199645713388,-20.7063083486775));
#38281=CARTESIAN_POINT('Ctrl Pts',(-16.6322706438836,17.7467356488663,-20.7106950655792));
#38282=CARTESIAN_POINT('Ctrl Pts',(-16.68499874854,17.6763359092247,-20.7150817824808));
#38283=CARTESIAN_POINT('Ctrl Pts',(-16.7377268531964,17.605936169583,-20.7194684993824));
#38284=CARTESIAN_POINT('Ctrl Pts',(-16.7940056129075,17.538366010084,-20.7238552162841));
#38285=CARTESIAN_POINT('Ctrl Pts',(-16.8534788424305,17.473979511942,-20.7282419331857));
#38286=CARTESIAN_POINT('Ctrl Pts',(-16.9102137543729,17.4125575523197,-20.7324266730952));
#38287=CARTESIAN_POINT('Ctrl Pts',(-16.970066659675,17.3538038607528,-20.7366114130047));
#38288=CARTESIAN_POINT('Ctrl Pts',(-17.0327566248197,17.2980517575206,-20.7407961529141));
#38289=CARTESIAN_POINT('Ctrl Pts',(-17.0953573508923,17.2423790173243,-20.7449749358526));
#38290=CARTESIAN_POINT('Ctrl Pts',(-17.1607867741654,17.189699681497,-20.749153718791));
#38291=CARTESIAN_POINT('Ctrl Pts',(-17.2287255995826,17.1403119550623,-20.7533325017295));
#38292=CARTESIAN_POINT('Ctrl Pts',(-17.2978800168063,17.0900405613692,-20.7575860533186));
#38293=CARTESIAN_POINT('Ctrl Pts',(-17.369634193181,17.0431800825081,-20.7618396049076));
#38294=CARTESIAN_POINT('Ctrl Pts',(-17.4436142556255,17.0000037017862,-20.7660931564967));
#38295=CARTESIAN_POINT('Ctrl Pts',(-17.516162301524,16.9576630772066,-20.7702643729802));
#38296=CARTESIAN_POINT('Ctrl Pts',(-17.5908504136365,16.9188654393416,-20.7744355894636));
#38297=CARTESIAN_POINT('Ctrl Pts',(-17.6672964027753,16.8838250096592,-20.7786068059471));
#38298=CARTESIAN_POINT('Ctrl Pts',(-17.7437167203783,16.8487963469989,-20.782776621683));
#38299=CARTESIAN_POINT('Ctrl Pts',(-17.8218933248018,16.8175225782417,-20.7869464374188));
#38300=CARTESIAN_POINT('Ctrl Pts',(-17.9014210276993,16.7901711636543,-20.7911162531547));
#38301=CARTESIAN_POINT('Ctrl Pts',(-17.980945877539,16.7628207302995,-20.7952859192984));
#38302=CARTESIAN_POINT('Ctrl Pts',(-18.0618212942028,16.7393925201402,-20.7994555854421));
#38303=CARTESIAN_POINT('Ctrl Pts',(-18.1436250863857,16.7200047247385,-20.8036252515858));
#38304=CARTESIAN_POINT('Ctrl Pts',(-18.2283005696263,16.6999363281423,-20.8079412922759));
#38305=CARTESIAN_POINT('Ctrl Pts',(-18.3139703091589,16.6841974227859,-20.812257332966));
#38306=CARTESIAN_POINT('Ctrl Pts',(-18.4001544252699,16.6728614828514,-20.8165733736561));
#38307=CARTESIAN_POINT('Ctrl Pts',(-18.4835353811664,16.6618942472358,-20.8207490340291));
#38308=CARTESIAN_POINT('Ctrl Pts',(-18.5673972928076,16.6550479436589,-20.8249246944022));
#38309=CARTESIAN_POINT('Ctrl Pts',(-18.6513021326319,16.6523360785885,-20.8291003547752));
#38310=CARTESIAN_POINT('Ctrl Pts',(-18.7394381312311,16.6494874594082,-20.8334865856239));
#38311=CARTESIAN_POINT('Ctrl Pts',(-18.8276209178941,16.651201212818,-20.8378728164725));
#38312=CARTESIAN_POINT('Ctrl Pts',(-18.915347159059,16.6574312799728,-20.8422590473212));
#38313=CARTESIAN_POINT('Ctrl Pts',(-19.0030734002238,16.6636613471276,-20.8466452781698));
#38314=CARTESIAN_POINT('Ctrl Pts',(-19.0903425295494,16.6744075817306,-20.8510315090185));
#38315=CARTESIAN_POINT('Ctrl Pts',(-19.1766642028218,16.6895622348469,-20.8554177398671));
#38316=CARTESIAN_POINT('Ctrl Pts',(-19.2590223527151,16.7040210508733,-20.859602573687));
#38317=CARTESIAN_POINT('Ctrl Pts',(-19.3408244952178,16.7225461130517,-20.8637874075069));
#38318=CARTESIAN_POINT('Ctrl Pts',(-19.4216382791443,16.7450815915656,-20.8679722413268));
#38319=CARTESIAN_POINT('Ctrl Pts',(-19.5023370763703,16.7675850052486,-20.8721511207141));
#38320=CARTESIAN_POINT('Ctrl Pts',(-19.5820498690826,16.7940873783027,-20.8763300001013));
#38321=CARTESIAN_POINT('Ctrl Pts',(-19.6603530717564,16.8244816182465,-20.8805088794886));
#38322=CARTESIAN_POINT('Ctrl Pts',(-19.7400550248591,16.8554187983856,-20.8847624072828));
#38323=CARTESIAN_POINT('Ctrl Pts',(-19.8182960576179,16.8903881737627,-20.8890159350769));
#38324=CARTESIAN_POINT('Ctrl Pts',(-19.8946441220389,16.9292232313444,-20.8932694628711));
#38325=CARTESIAN_POINT('Ctrl Pts',(-19.9695165810175,16.9673077103389,-20.8974407812627));
#38326=CARTESIAN_POINT('Ctrl Pts',(-20.0425681641198,17.0091095557736,-20.9016120996543));
#38327=CARTESIAN_POINT('Ctrl Pts',(-20.1134118643462,17.0544233358165,-20.9057834180459));
#38328=CARTESIAN_POINT('Ctrl Pts',(-20.1842318054818,17.0997219188241,-20.9099533374884));
#38329=CARTESIAN_POINT('Ctrl Pts',(-20.2528449471495,17.1485298496365,-20.9141232569308));
#38330=CARTESIAN_POINT('Ctrl Pts',(-20.3188911542421,17.2005970480511,-20.9182931763733));
#38331=CARTESIAN_POINT('Ctrl Pts',(-20.3849350181168,17.2526623992014,-20.9224629478734));
#38332=CARTESIAN_POINT('Ctrl Pts',(-20.4484117677876,17.3079865025997,-20.9266327193736));
#38333=CARTESIAN_POINT('Ctrl Pts',(-20.5089934936092,17.3662783143127,-20.9308024908737));
#38334=CARTESIAN_POINT('Ctrl Pts',(-20.5716985989688,17.4266132444504,-20.9351184121799));
#38335=CARTESIAN_POINT('Ctrl Pts',(-20.6313015884267,17.4901274194612,-20.9394343334862));
#38336=CARTESIAN_POINT('Ctrl Pts',(-20.6874809779159,17.5564571420115,-20.9437502547924));
#38337=CARTESIAN_POINT('Ctrl Pts',(-20.7418360321656,17.6206329135956,-20.9479260235017));
#38338=CARTESIAN_POINT('Ctrl Pts',(-20.7929861867181,17.6874437676866,-20.9521017922111));
#38339=CARTESIAN_POINT('Ctrl Pts',(-20.84068298328,17.756528684381,-20.9562775609204));
#38340=CARTESIAN_POINT('Ctrl Pts',(-20.8907810730051,17.8290916782231,-20.9606635585251));
#38341=CARTESIAN_POINT('Ctrl Pts',(-20.937068653801,17.9041632231128,-20.9650495561297));
#38342=CARTESIAN_POINT('Ctrl Pts',(-20.9793120563336,17.9812952510122,-20.9694355537344));
#38343=CARTESIAN_POINT('Ctrl Pts',(-21.0215554588661,18.0584272789116,-20.9738215513391));
#38344=CARTESIAN_POINT('Ctrl Pts',(-21.0597544996862,18.1376192346801,-20.9782075489438));
#38345=CARTESIAN_POINT('Ctrl Pts',(-21.0937343932684,18.2184005877363,-20.9825935465485));
#38346=CARTESIAN_POINT('Ctrl Pts',(-21.1297845102027,18.3041035407708,-20.9872467608424));
#38347=CARTESIAN_POINT('Ctrl Pts',(-21.1612011557346,18.3918658581185,-20.9918999751363));
#38348=CARTESIAN_POINT('Ctrl Pts',(-21.1877704304992,18.4811981951189,-20.9965531894303));
#38349=CARTESIAN_POINT('Ctrl Pts',(-21.2142564917145,18.5702507480116,-21.0011918301056));
#38350=CARTESIAN_POINT('Ctrl Pts',(-21.2359253488098,18.6608632602714,-21.0058304707809));
#38351=CARTESIAN_POINT('Ctrl Pts',(-21.2526114411354,18.7525281812567,-21.0104691114562));
#38352=CARTESIAN_POINT('Ctrl Pts',(-21.2692072331732,18.8436970382994,-21.0150826491548));
#38353=CARTESIAN_POINT('Ctrl Pts',(-21.2808739262263,18.9359066855585,-21.0196961868533));
#38354=CARTESIAN_POINT('Ctrl Pts',(-21.2874965126302,19.0286389296337,-21.0243097245519));
#38355=CARTESIAN_POINT('Ctrl Pts',(-21.2917935179279,19.0888074075896,-21.0273031767656));
#38356=CARTESIAN_POINT('Ctrl Pts',(-21.2939679583765,19.1491955214723,-21.0302966289794));
#38357=CARTESIAN_POINT('Ctrl Pts',(-21.2939996483756,19.2096582411964,-21.0332900811932));
#38358=CARTESIAN_POINT('Ctrl Pts',(-21.2904840295148,19.2096606602608,-21.0332901097715));
#38359=CARTESIAN_POINT('Ctrl Pts',(-21.288030249326,19.7238724906044,-21.0587831909243));
#38360=CARTESIAN_POINT('Ctrl Pts',(-20.8878309688531,21.0966582904734,-21.1266682076376));
#38361=CARTESIAN_POINT('Ctrl Pts',(-18.9689508715201,22.0730071282985,-21.2211092990968));
#38362=CARTESIAN_POINT('Ctrl Pts',(-17.6030346275064,21.5621391285562,-21.2900573094031));
#38363=CARTESIAN_POINT('Ctrl Pts',(-17.1763093513331,21.2386979557192,-21.3166133841489));
#38364=CARTESIAN_POINT('',(-21.2964371679699,19.2128544327287,-20.9667098902285));
#38365=CARTESIAN_POINT('Ctrl Pts',(-21.2964371679699,19.2128544327287,-20.9667098902285));
#38366=CARTESIAN_POINT('Ctrl Pts',(-21.2973789664463,19.3284704701528,-20.9724759609646));
#38367=CARTESIAN_POINT('Ctrl Pts',(-21.2376963737069,20.2931122040567,-21.0206339672611));
#38368=CARTESIAN_POINT('Ctrl Pts',(-20.0126665865687,21.9547543377114,-21.1111839091181));
#38369=CARTESIAN_POINT('Ctrl Pts',(-17.9939164834006,21.8268016750118,-21.1999086048959));
#38370=CARTESIAN_POINT('Ctrl Pts',(-17.2346906284817,21.2922910373603,-21.2462413651133));
#38371=CARTESIAN_POINT('Ctrl Pts',(-17.1724222554293,21.243756036567,-21.2501821897702));
#38372=CARTESIAN_POINT('Ctrl Pts',(-17.1739275520481,21.2418454004355,-20.4499991710565));
#38373=CARTESIAN_POINT('Ctrl Pts',(-17.0385457538407,21.1400081684298,-20.4584344059413));
#38374=CARTESIAN_POINT('Ctrl Pts',(-16.2862201916857,20.4464549384029,-20.5092615763866));
#38375=CARTESIAN_POINT('Ctrl Pts',(-15.8255860927207,18.3717008434114,-20.6024806823924));
#38376=CARTESIAN_POINT('Ctrl Pts',(-17.8654473830542,16.3111912047089,-20.7296564890738));
#38377=CARTESIAN_POINT('Ctrl Pts',(-20.5735369877998,16.8838680312786,-20.8510662250192));
#38378=CARTESIAN_POINT('Ctrl Pts',(-21.2904548994085,18.4784657038926,-20.9300840254041));
#38379=CARTESIAN_POINT('Ctrl Pts',(-21.2964371679699,19.2128544327287,-20.9667098902285));
#38380=CARTESIAN_POINT('Origin',(-18.734,19.211,1.76670989022852));
#38381=CARTESIAN_POINT('',(-17.1744642439897,21.2411350264762,-19.6501081077316));
#38382=CARTESIAN_POINT('',(-17.1744642439897,21.2411350264762,-19.7167245443048));
#38383=CARTESIAN_POINT('',(-17.1744642439897,21.2411350264762,1.76670989022852));
#38384=CARTESIAN_POINT('',(-21.2939995273706,19.2094444092821,-20.2332901098006));
#38385=CARTESIAN_POINT('Ctrl Pts',(-17.1744642439897,21.2411350264762,-19.7167245443048));
#38386=CARTESIAN_POINT('Ctrl Pts',(-17.1080940647866,21.1901499115699,-19.7209062128092));
#38387=CARTESIAN_POINT('Ctrl Pts',(-17.0441149697057,21.1358207858829,-19.7250878813135));
#38388=CARTESIAN_POINT('Ctrl Pts',(-16.982882251611,21.0784010365417,-19.7292695498179));
#38389=CARTESIAN_POINT('Ctrl Pts',(-16.9217271760624,21.0210540949359,-19.7334459160035));
#38390=CARTESIAN_POINT('Ctrl Pts',(-16.8633118927493,20.9606246273613,-19.7376222821892));
#38391=CARTESIAN_POINT('Ctrl Pts',(-16.8079596809234,20.8974070354725,-19.7417986483748));
#38392=CARTESIAN_POINT('Ctrl Pts',(-16.7526597829306,20.8342491910526,-19.7459710674422));
#38393=CARTESIAN_POINT('Ctrl Pts',(-16.7004175050121,20.7683088038869,-19.7501434865096));
#38394=CARTESIAN_POINT('Ctrl Pts',(-16.6515192476679,20.6999170279657,-19.754315905577));
#38395=CARTESIAN_POINT('Ctrl Pts',(-16.60264546862,20.6315594887279,-19.758486235946));
#38396=CARTESIAN_POINT('Ctrl Pts',(-16.5571126534136,20.5607533708702,-19.7626565663151));
#38397=CARTESIAN_POINT('Ctrl Pts',(-16.5151661257008,20.487861871254,-19.7668268966841));
#38398=CARTESIAN_POINT('Ctrl Pts',(-16.4732280132432,20.4149849950311,-19.7709963904071));
#38399=CARTESIAN_POINT('Ctrl Pts',(-16.4348749882279,20.3400239668443,-19.7751658841302));
#38400=CARTESIAN_POINT('Ctrl Pts',(-16.4003076097238,20.2633686747366,-19.7793353778532));
#38401=CARTESIAN_POINT('Ctrl Pts',(-16.365736796812,20.1867057666183,-19.7835052858322));
#38402=CARTESIAN_POINT('Ctrl Pts',(-16.3349525651543,20.1083486802376,-19.7876751938112));
#38403=CARTESIAN_POINT('Ctrl Pts',(-16.3081077362453,20.0287082148634,-19.7918451017901));
#38404=CARTESIAN_POINT('Ctrl Pts',(-16.2812344363892,19.948983284824,-19.7960194322681));
#38405=CARTESIAN_POINT('Ctrl Pts',(-16.2583090282375,19.8679726950072,-19.8001937627461));
#38406=CARTESIAN_POINT('Ctrl Pts',(-16.2394345742077,19.7861028920479,-19.8043680932241));
#38407=CARTESIAN_POINT('Ctrl Pts',(-16.2205495154889,19.7041870902052,-19.8085447690667));
#38408=CARTESIAN_POINT('Ctrl Pts',(-16.2057200237114,19.6214115669634,-19.8127214449094));
#38409=CARTESIAN_POINT('Ctrl Pts',(-16.194997652802,19.5382110647933,-19.816898120752));
#38410=CARTESIAN_POINT('Ctrl Pts',(-16.1842568910067,19.4548678580888,-19.8210819603805));
#38411=CARTESIAN_POINT('Ctrl Pts',(-16.1776373544537,19.3710986755521,-19.825265800009));
#38412=CARTESIAN_POINT('Ctrl Pts',(-16.1751385298197,19.2873411843422,-19.8294496396375));
#38413=CARTESIAN_POINT('Ctrl Pts',(-16.1734340306215,19.230208492968,-19.8323035218969));
#38414=CARTESIAN_POINT('Ctrl Pts',(-16.1736457558925,19.1730812523769,-19.8351574041563));
#38415=CARTESIAN_POINT('Ctrl Pts',(-16.1757597065464,19.1160968865085,-19.8380112864156));
#38416=CARTESIAN_POINT('Ctrl Pts',(-16.1788593811049,19.0325410150462,-19.8421959187372));
#38417=CARTESIAN_POINT('Ctrl Pts',(-16.1860627143394,18.9489816683593,-19.8463805510587));
#38418=CARTESIAN_POINT('Ctrl Pts',(-16.1973733531866,18.8658547339507,-19.8505651833802));
#38419=CARTESIAN_POINT('Ctrl Pts',(-16.2086678927321,18.7828461204975,-19.8547438593928));
#38420=CARTESIAN_POINT('Ctrl Pts',(-16.2240580639186,18.700269148709,-19.8589225354055));
#38421=CARTESIAN_POINT('Ctrl Pts',(-16.2434955346196,18.6185580130341,-19.8631012114182));
#38422=CARTESIAN_POINT('Ctrl Pts',(-16.2632814202296,18.5353822126226,-19.8673547898215));
#38423=CARTESIAN_POINT('Ctrl Pts',(-16.287261115507,18.4531040767777,-19.8716083682248));
#38424=CARTESIAN_POINT('Ctrl Pts',(-16.315328555729,18.3721743657541,-19.875861946628));
#38425=CARTESIAN_POINT('Ctrl Pts',(-16.3428518369366,18.2928136838773,-19.8800330585501));
#38426=CARTESIAN_POINT('Ctrl Pts',(-16.3743056171544,18.2147500627578,-19.8842041704722));
#38427=CARTESIAN_POINT('Ctrl Pts',(-16.4095391529049,18.1383948674737,-19.8883752823943));
#38428=CARTESIAN_POINT('Ctrl Pts',(-16.4447608657818,18.0620652937402,-19.8925449946689));
#38429=CARTESIAN_POINT('Ctrl Pts',(-16.4837596226908,17.9874434246684,-19.8967147069435));
#38430=CARTESIAN_POINT('Ctrl Pts',(-16.5263367853317,17.9149200909664,-19.9008844192181));
#38431=CARTESIAN_POINT('Ctrl Pts',(-16.5689124330239,17.8423993377355,-19.9050539831292));
#38432=CARTESIAN_POINT('Ctrl Pts',(-16.6150659996536,17.7719773677011,-19.9092235470402));
#38433=CARTESIAN_POINT('Ctrl Pts',(-16.6645538728597,17.7040186706983,-19.9133931109512));
#38434=CARTESIAN_POINT('Ctrl Pts',(-16.7157817325743,17.6336705556774,-19.9177092761301));
#38435=CARTESIAN_POINT('Ctrl Pts',(-16.7705824268663,17.5659625858456,-19.9220254413089));
#38436=CARTESIAN_POINT('Ctrl Pts',(-16.828639391307,17.5012629000805,-19.9263416064877));
#38437=CARTESIAN_POINT('Ctrl Pts',(-16.8848050978436,17.4386708648494,-19.9305171686985));
#38438=CARTESIAN_POINT('Ctrl Pts',(-16.9440178150289,17.3788944293155,-19.9346927309094));
#38439=CARTESIAN_POINT('Ctrl Pts',(-17.0059537750657,17.3222289062752,-19.9388682931203));
#38440=CARTESIAN_POINT('Ctrl Pts',(-17.0710180730474,17.2627012510296,-19.9432547597831));
#38441=CARTESIAN_POINT('Ctrl Pts',(-17.1390875043195,17.2066074135524,-19.9476412264458));
#38442=CARTESIAN_POINT('Ctrl Pts',(-17.2097498587669,17.154240046347,-19.9520276931086));
#38443=CARTESIAN_POINT('Ctrl Pts',(-17.2804122132143,17.1018726791415,-19.9564141597714));
#38444=CARTESIAN_POINT('Ctrl Pts',(-17.3536669653909,17.0532320397927,-19.9608006264342));
#38445=CARTESIAN_POINT('Ctrl Pts',(-17.4290716121177,17.0085554711869,-19.965187093097));
#38446=CARTESIAN_POINT('Ctrl Pts',(-17.501006718607,16.9659345736727,-19.9693717283973));
#38447=CARTESIAN_POINT('Ctrl Pts',(-17.5751659817943,16.9267623274508,-19.9735563636976));
#38448=CARTESIAN_POINT('Ctrl Pts',(-17.6511848627828,16.8912777367509,-19.9777409989979));
#38449=CARTESIAN_POINT('Ctrl Pts',(-17.7270955400278,16.8558436541026,-19.9819196779726));
#38450=CARTESIAN_POINT('Ctrl Pts',(-17.8048601641239,16.8240869938583,-19.9860983569473));
#38451=CARTESIAN_POINT('Ctrl Pts',(-17.8840874845046,16.7962021376512,-19.990277035922));
#38452=CARTESIAN_POINT('Ctrl Pts',(-17.9647348762106,16.7678174729877,-19.9945306135827));
#38453=CARTESIAN_POINT('Ctrl Pts',(-18.0468975020319,16.7434450254351,-19.9987841912434));
#38454=CARTESIAN_POINT('Ctrl Pts',(-18.1301389337681,16.723239599019,-20.0030377689041));
#38455=CARTESIAN_POINT('Ctrl Pts',(-18.2117665887585,16.7034258891629,-20.0072088837266));
#38456=CARTESIAN_POINT('Ctrl Pts',(-18.2944311263188,16.6876191861686,-20.0113799985491));
#38457=CARTESIAN_POINT('Ctrl Pts',(-18.3777050584842,16.6759154028612,-20.0155511133716));
#38458=CARTESIAN_POINT('Ctrl Pts',(-18.4609510469055,16.6642155469237,-20.0197208285176));
#38459=CARTESIAN_POINT('Ctrl Pts',(-18.5448055686334,16.6566159403141,-20.0238905436636));
#38460=CARTESIAN_POINT('Ctrl Pts',(-18.6288324772911,16.6531611090283,-20.0280602588096));
#38461=CARTESIAN_POINT('Ctrl Pts',(-18.7128563955109,16.6497064006967,-20.0322298255595));
#38462=CARTESIAN_POINT('Ctrl Pts',(-18.7970522287831,16.6503961924512,-20.0363993923093));
#38463=CARTESIAN_POINT('Ctrl Pts',(-18.880981635612,16.6552229364061,-20.0405689590591));
#38464=CARTESIAN_POINT('Ctrl Pts',(-18.9678618596805,16.6602193805865,-20.0448851207857));
#38465=CARTESIAN_POINT('Ctrl Pts',(-19.0544560473056,16.6696490660325,-20.0492012825123));
#38466=CARTESIAN_POINT('Ctrl Pts',(-19.1402833031872,16.6834450792216,-20.0535174442389));
#38467=CARTESIAN_POINT('Ctrl Pts',(-19.2233147795964,16.6967916942552,-20.0576930091793));
#38468=CARTESIAN_POINT('Ctrl Pts',(-19.3056280709207,16.7142243988718,-20.0618685741196));
#38469=CARTESIAN_POINT('Ctrl Pts',(-19.3867996159112,16.735630802998,-20.0660441390599));
#38470=CARTESIAN_POINT('Ctrl Pts',(-19.4720708905892,16.7581183799726,-20.0704305991796));
#38471=CARTESIAN_POINT('Ctrl Pts',(-19.5560814939681,16.7849914459207,-20.0748170592994));
#38472=CARTESIAN_POINT('Ctrl Pts',(-19.6383622323597,16.8160618060832,-20.0792035194192));
#38473=CARTESIAN_POINT('Ctrl Pts',(-19.7206429707512,16.8471321662457,-20.0835899795389));
#38474=CARTESIAN_POINT('Ctrl Pts',(-19.8011933431587,16.8823995182362,-20.0879764396587));
#38475=CARTESIAN_POINT('Ctrl Pts',(-19.8795742651096,16.9216202579916,-20.0923628997785));
#38476=CARTESIAN_POINT('Ctrl Pts',(-19.9543489005549,16.9590364613751,-20.0965475399714));
#38477=CARTESIAN_POINT('Ctrl Pts',(-20.0274276526341,17.0001895262269,-20.1007321801642));
#38478=CARTESIAN_POINT('Ctrl Pts',(-20.0984122381085,17.0449023003337,-20.1049168203571));
#38479=CARTESIAN_POINT('Ctrl Pts',(-20.1692957865176,17.0895514317855,-20.1090955042742));
#38480=CARTESIAN_POINT('Ctrl Pts',(-20.2380907031438,17.137749965204,-20.1132741881914));
#38481=CARTESIAN_POINT('Ctrl Pts',(-20.3044217668728,17.189274134772,-20.1174528721085));
#38482=CARTESIAN_POINT('Ctrl Pts',(-20.3719416499117,17.2417217469061,-20.1217064485398));
#38483=CARTESIAN_POINT('Ctrl Pts',(-20.4369080598406,17.2976151641855,-20.1259600249711));
#38484=CARTESIAN_POINT('Ctrl Pts',(-20.4989546019222,17.3566712122297,-20.1302136014024));
#38485=CARTESIAN_POINT('Ctrl Pts',(-20.5597983571728,17.4145824448741,-20.1343847212528));
#38486=CARTESIAN_POINT('Ctrl Pts',(-20.6178340905372,17.4755344539392,-20.1385558411033));
#38487=CARTESIAN_POINT('Ctrl Pts',(-20.6727497630573,17.5392197045529,-20.1427269609537));
#38488=CARTESIAN_POINT('Ctrl Pts',(-20.7276470081433,17.6028835850239,-20.1468966811484));
#38489=CARTESIAN_POINT('Ctrl Pts',(-20.7794259715033,17.6692785374397,-20.151066401343));
#38490=CARTESIAN_POINT('Ctrl Pts',(-20.8278131357729,17.7380619318977,-20.1552361215377));
#38491=CARTESIAN_POINT('Ctrl Pts',(-20.8761985781537,17.8068428786539,-20.1594056933502));
#38492=CARTESIAN_POINT('Ctrl Pts',(-20.9211921974361,17.8780117217137,-20.1635752651627));
#38493=CARTESIAN_POINT('Ctrl Pts',(-20.9625630739946,17.9511957988531,-20.1677448369751));
#38494=CARTESIAN_POINT('Ctrl Pts',(-21.0053883703184,18.0269527092786,-20.1720609927655));
#38495=CARTESIAN_POINT('Ctrl Pts',(-21.0443311966684,18.104868729537,-20.1763771485559));
#38496=CARTESIAN_POINT('Ctrl Pts',(-21.0791875184544,18.1845032862763,-20.1806933043463));
#38497=CARTESIAN_POINT('Ctrl Pts',(-21.112908500301,18.2615439866305,-20.1848688743318));
#38498=CARTESIAN_POINT('Ctrl Pts',(-21.1428049786358,18.3401925327768,-20.1890444443173));
#38499=CARTESIAN_POINT('Ctrl Pts',(-21.1687421896672,18.4200319413184,-20.1932200143028));
#38500=CARTESIAN_POINT('Ctrl Pts',(-21.1959893070235,18.5039034775277,-20.1976064629957));
#38501=CARTESIAN_POINT('Ctrl Pts',(-21.2188665678873,18.5890887630882,-20.2019929116885));
#38502=CARTESIAN_POINT('Ctrl Pts',(-21.2372782491424,18.6750914188312,-20.2063793603814));
#38503=CARTESIAN_POINT('Ctrl Pts',(-21.2556899303975,18.7610940745742,-20.2107658090742));
#38504=CARTESIAN_POINT('Ctrl Pts',(-21.2696360151223,18.8479135155775,-20.215152257767));
#38505=CARTESIAN_POINT('Ctrl Pts',(-21.2790836672405,18.935048687726,-20.2195387064599));
#38506=CARTESIAN_POINT('Ctrl Pts',(-21.288956382332,19.0261041921328,-20.2241225075637));
#38507=CARTESIAN_POINT('Ctrl Pts',(-21.2939437779116,19.1176988534549,-20.2287063086676));
#38508=CARTESIAN_POINT('Ctrl Pts',(-21.2939995273702,19.2094444086991,-20.2332901097715));
#38509=CARTESIAN_POINT('Ctrl Pts',(-21.2939995273706,19.209444409282,-20.2332901098006));
#38510=CARTESIAN_POINT('Ctrl Pts',(-21.2940497238898,19.292051655634,-20.2374173417521));
#38511=CARTESIAN_POINT('Ctrl Pts',(-21.2900972916445,19.3748187808655,-20.2415445737036));
#38512=CARTESIAN_POINT('Ctrl Pts',(-21.2821221995875,19.4573194185792,-20.2456718056551));
#38513=CARTESIAN_POINT('Ctrl Pts',(-21.2739869560054,19.5414767898907,-20.249881918467));
#38514=CARTESIAN_POINT('Ctrl Pts',(-21.2616656478282,19.6253563615795,-20.254092031279));
#38515=CARTESIAN_POINT('Ctrl Pts',(-21.2451929662144,19.7085036546953,-20.2583021440909));
#38516=CARTESIAN_POINT('Ctrl Pts',(-21.2290800677258,19.7898349111956,-20.262420302989));
#38517=CARTESIAN_POINT('Ctrl Pts',(-21.2089953889688,19.8704650608503,-20.2665384618872));
#38518=CARTESIAN_POINT('Ctrl Pts',(-21.1850236968841,19.9499741790566,-20.2706566207853));
#38519=CARTESIAN_POINT('Ctrl Pts',(-21.1610629739661,20.0294469148178,-20.274772895262));
#38520=CARTESIAN_POINT('Ctrl Pts',(-21.1332189034159,20.1077991846501,-20.2788891697386));
#38521=CARTESIAN_POINT('Ctrl Pts',(-21.1016267106028,20.1846240338243,-20.2830054442153));
#38522=CARTESIAN_POINT('Ctrl Pts',(-21.0700389112288,20.2614381991786,-20.287121146253));
#38523=CARTESIAN_POINT('Ctrl Pts',(-21.0347042052762,20.3367249283834,-20.2912368482907));
#38524=CARTESIAN_POINT('Ctrl Pts',(-20.9958062168364,20.4100965922228,-20.2953525503285));
#38525=CARTESIAN_POINT('Ctrl Pts',(-20.9553538829569,20.4864001534601,-20.2996327138962));
#38526=CARTESIAN_POINT('Ctrl Pts',(-20.9110477401698,20.5606318825454,-20.3039128774639));
#38527=CARTESIAN_POINT('Ctrl Pts',(-20.8631463404351,20.6323851909359,-20.3081930410317));
#38528=CARTESIAN_POINT('Ctrl Pts',(-20.8170263796525,20.7014700149142,-20.3123140265766));
#38529=CARTESIAN_POINT('Ctrl Pts',(-20.7675741880587,20.7682571483522,-20.3164350121215));
#38530=CARTESIAN_POINT('Ctrl Pts',(-20.7150628498031,20.832416043195,-20.3205559976664));
#38531=CARTESIAN_POINT('Ctrl Pts',(-20.6625158670912,20.8966184888021,-20.3246797805174));
#38532=CARTESIAN_POINT('Ctrl Pts',(-20.6069059263909,20.958188799342,-20.3288035633684));
#38533=CARTESIAN_POINT('Ctrl Pts',(-20.5485433933874,21.0168328476119,-20.3329273462195));
#38534=CARTESIAN_POINT('Ctrl Pts',(-20.4900913059675,21.0755668822695,-20.3370574568111));
#38535=CARTESIAN_POINT('Ctrl Pts',(-20.4288785557237,21.1313653881747,-20.3411875674027));
#38536=CARTESIAN_POINT('Ctrl Pts',(-20.3652483070037,21.1839746478091,-20.3453176779943));
#38537=CARTESIAN_POINT('Ctrl Pts',(-20.358074893939,21.1899055998009,-20.3457832897099));
#38538=CARTESIAN_POINT('Ctrl Pts',(-20.3508707850611,21.1957960645337,-20.3462489014256));
#38539=CARTESIAN_POINT('Ctrl Pts',(-20.3436364935458,21.2016457139947,-20.3467145131413));
#38540=CARTESIAN_POINT('Ctrl Pts',(-20.278618922688,21.2542189338493,-20.3508991582656));
#38541=CARTESIAN_POINT('Ctrl Pts',(-20.2109019654201,21.3037012778441,-20.3550838033898));
#38542=CARTESIAN_POINT('Ctrl Pts',(-20.1408117781385,21.3498035489242,-20.3592684485141));
#38543=CARTESIAN_POINT('Ctrl Pts',(-20.0708213570877,21.3958401981249,-20.363447137223));
#38544=CARTESIAN_POINT('Ctrl Pts',(-19.9984647969503,21.4385060803064,-20.3676258259318));
#38545=CARTESIAN_POINT('Ctrl Pts',(-19.9241011364255,21.4775522903915,-20.3718045146407));
#38546=CARTESIAN_POINT('Ctrl Pts',(-19.8484048007058,21.5172982497259,-20.3760580898566));
#38547=CARTESIAN_POINT('Ctrl Pts',(-19.770629090414,21.553293216013,-20.3803116650725));
#38548=CARTESIAN_POINT('Ctrl Pts',(-19.6911834656509,21.5853209161957,-20.3845652402884));
#38549=CARTESIAN_POINT('Ctrl Pts',(-19.6132778082299,21.6167277941183,-20.3887363645583));
#38550=CARTESIAN_POINT('Ctrl Pts',(-19.5337668439882,21.6443196560401,-20.3929074888282));
#38551=CARTESIAN_POINT('Ctrl Pts',(-19.4530597043387,21.6679397920169,-20.3970786130981));
#38552=CARTESIAN_POINT('Ctrl Pts',(-19.3723796494948,21.6915520012256,-20.4012483375651));
#38553=CARTESIAN_POINT('Ctrl Pts',(-19.2905046576304,21.7111950025156,-20.4054180620321));
#38554=CARTESIAN_POINT('Ctrl Pts',(-19.2078598569048,21.7267616810847,-20.409587786499));
#38555=CARTESIAN_POINT('Ctrl Pts',(-19.1252180001541,21.7423278051372,-20.413757362432));
#38556=CARTESIAN_POINT('Ctrl Pts',(-19.041806841303,21.7538178108621,-20.4179269383649));
#38557=CARTESIAN_POINT('Ctrl Pts',(-18.9580612092296,21.7611757928658,-20.4220965142979));
#38558=CARTESIAN_POINT('Ctrl Pts',(-18.8713716383372,21.7687924325249,-20.4264126647583));
#38559=CARTESIAN_POINT('Ctrl Pts',(-18.7843241655966,21.7719810786356,-20.4307288152187));
#38560=CARTESIAN_POINT('Ctrl Pts',(-18.6974043027305,21.7707384153349,-20.4350449656791));
#38561=CARTESIAN_POINT('Ctrl Pts',(-18.6133154147563,21.7695362255058,-20.4392205393694));
#38562=CARTESIAN_POINT('Ctrl Pts',(-18.5293464188554,21.7641870271194,-20.4433961130596));
#38563=CARTESIAN_POINT('Ctrl Pts',(-18.4459326767642,21.7547407920784,-20.4475716867499));
#38564=CARTESIAN_POINT('Ctrl Pts',(-18.3583065669894,21.7448175251453,-20.4519581255954));
#38565=CARTESIAN_POINT('Ctrl Pts',(-18.271293843584,21.7303726259075,-20.4563445644409));
#38566=CARTESIAN_POINT('Ctrl Pts',(-18.1853859711597,21.7115244744572,-20.4607310032864));
#38567=CARTESIAN_POINT('Ctrl Pts',(-18.0994780987354,21.6926763230069,-20.4651174421318));
#38568=CARTESIAN_POINT('Ctrl Pts',(-18.0146756167236,21.6694251461087,-20.4695038809773));
#38569=CARTESIAN_POINT('Ctrl Pts',(-17.9314482086413,21.6419485025781,-20.4738903198228));
#38570=CARTESIAN_POINT('Ctrl Pts',(-17.8520649990632,21.6157409802949,-20.4780741530359));
#38571=CARTESIAN_POINT('Ctrl Pts',(-17.7738191779357,21.5855921988556,-20.4822579862489));
#38572=CARTESIAN_POINT('Ctrl Pts',(-17.6971302094549,21.5516197977149,-20.486441819462));
#38573=CARTESIAN_POINT('Ctrl Pts',(-17.6205369358846,21.5176897884064,-20.4906204319562));
#38574=CARTESIAN_POINT('Ctrl Pts',(-17.545497076438,21.4799458123768,-20.4947990444504));
#38575=CARTESIAN_POINT('Ctrl Pts',(-17.4724142389696,21.4385550200984,-20.4989776569446));
#38576=CARTESIAN_POINT('Ctrl Pts',(-17.3994143840766,21.397211225373,-20.503151524795));
#38577=CARTESIAN_POINT('Ctrl Pts',(-17.3283675330366,21.3522290693436,-20.5073253926455));
#38578=CARTESIAN_POINT('Ctrl Pts',(-17.2596551457062,21.3038227948437,-20.511499260496));
#38579=CARTESIAN_POINT('Ctrl Pts',(-17.2308389678685,21.2835224695509,-20.5132496714906));
#38580=CARTESIAN_POINT('Ctrl Pts',(-17.2024330747213,21.2626204897635,-20.5150000824852));
#38581=CARTESIAN_POINT('Ctrl Pts',(-17.1744642439897,21.2411350264762,-20.5167504934799));
#38582=CARTESIAN_POINT('',(-21.2937660450662,19.2120076676442,-20.1667099326));
#38583=CARTESIAN_POINT('Ctrl Pts',(-21.2901594272135,19.212019439545,-20.166710586346));
#38584=CARTESIAN_POINT('Ctrl Pts',(-21.2914431884923,19.5768333887026,-20.1847914783466));
#38585=CARTESIAN_POINT('Ctrl Pts',(-21.0477248310816,20.7953392166858,-20.2452643059079));
#38586=CARTESIAN_POINT('Ctrl Pts',(-19.3278236771125,22.0902445830675,-20.3396938341447));
#38587=CARTESIAN_POINT('Ctrl Pts',(-17.7189176159228,21.6517991779038,-20.4160424703808));
#38588=CARTESIAN_POINT('Ctrl Pts',(-17.1739275520481,21.2418454004355,-20.4499991710565));
#38589=CARTESIAN_POINT('Ctrl Pts',(-17.1744642439897,21.2411350264762,-19.6501081077317));
#38590=CARTESIAN_POINT('Ctrl Pts',(-17.1077738078371,21.1899038923853,-19.6542777748744));
#38591=CARTESIAN_POINT('Ctrl Pts',(-17.0436134208209,21.135385404573,-19.6584474420171));
#38592=CARTESIAN_POINT('Ctrl Pts',(-16.9823135556347,21.0778675905449,-19.6626171091599));
#38593=CARTESIAN_POINT('Ctrl Pts',(-16.9209517695699,21.0202916760043,-19.6667909882116));
#38594=CARTESIAN_POINT('Ctrl Pts',(-16.8624566135658,20.9597106987123,-19.6709648672633));
#38595=CARTESIAN_POINT('Ctrl Pts',(-16.8071223925888,20.8964502917788,-19.675138746315));
#38596=CARTESIAN_POINT('Ctrl Pts',(-16.7517612063089,20.8331590569777,-19.6793146593687));
#38597=CARTESIAN_POINT('Ctrl Pts',(-16.6995643093342,20.7671861526635,-19.6834905724224));
#38598=CARTESIAN_POINT('Ctrl Pts',(-16.6507847507581,20.6988891844912,-19.687666485476));
#38599=CARTESIAN_POINT('Ctrl Pts',(-16.6019172419757,20.6304690759582,-19.6918499277576));
#38600=CARTESIAN_POINT('Ctrl Pts',(-16.5564796329369,20.5597169183466,-19.6960333700392));
#38601=CARTESIAN_POINT('Ctrl Pts',(-16.5146807414217,20.4870180361199,-19.7002168123208));
#38602=CARTESIAN_POINT('Ctrl Pts',(-16.4746040644093,20.4173145220662,-19.7042278867546));
#38603=CARTESIAN_POINT('Ctrl Pts',(-16.4378722674183,20.3458218948274,-19.7082389611885));
#38604=CARTESIAN_POINT('Ctrl Pts',(-16.4046276535517,20.2728966388503,-19.7122500356223));
#38605=CARTESIAN_POINT('Ctrl Pts',(-16.3699445411192,20.1968158980013,-19.7164346697445));
#38606=CARTESIAN_POINT('Ctrl Pts',(-16.3389281684758,20.1188925846309,-19.7206193038666));
#38607=CARTESIAN_POINT('Ctrl Pts',(-16.3117771822155,20.0395147077776,-19.7248039379887));
#38608=CARTESIAN_POINT('Ctrl Pts',(-16.2846648420244,19.9602498155099,-19.728982615802));
#38609=CARTESIAN_POINT('Ctrl Pts',(-16.2614071073244,19.879534903759,-19.7331612936152));
#38610=CARTESIAN_POINT('Ctrl Pts',(-16.2421554012761,19.797779767724,-19.7373399714285));
#38611=CARTESIAN_POINT('Ctrl Pts',(-16.2225586206514,19.7145592229166,-19.7415935493816));
#38612=CARTESIAN_POINT('Ctrl Pts',(-16.2071130980707,19.6302612335116,-19.7458471273348));
#38613=CARTESIAN_POINT('Ctrl Pts',(-16.1959260745095,19.5453362809288,-19.7501007052879));
#38614=CARTESIAN_POINT('Ctrl Pts',(-16.1849559341096,19.4620577709489,-19.7542718189977));
#38615=CARTESIAN_POINT('Ctrl Pts',(-16.1780807097821,19.3781768678582,-19.7584429327075));
#38616=CARTESIAN_POINT('Ctrl Pts',(-16.175350045093,19.294128865351,-19.7626140464172));
#38617=CARTESIAN_POINT('Ctrl Pts',(-16.172620296704,19.2101090659343,-19.766783760471));
#38618=CARTESIAN_POINT('Ctrl Pts',(-16.1740323608365,19.1259227378681,-19.7709534745247));
#38619=CARTESIAN_POINT('Ctrl Pts',(-16.1795838629489,19.0420082878574,-19.7751231885784));
#38620=CARTESIAN_POINT('Ctrl Pts',(-16.1851351675175,18.9580968238458,-19.7792927542576));
#38621=CARTESIAN_POINT('Ctrl Pts',(-16.1948255859832,18.8744576776277,-19.7834623199368));
#38622=CARTESIAN_POINT('Ctrl Pts',(-16.2086007338245,18.7915258692122,-19.787631885616));
#38623=CARTESIAN_POINT('Ctrl Pts',(-16.2228602008279,18.7056782689351,-19.7919480486733));
#38624=CARTESIAN_POINT('Ctrl Pts',(-16.2414968944959,18.6205891924187,-19.7962642117307));
#38625=CARTESIAN_POINT('Ctrl Pts',(-16.2643928538834,18.536729621109,-19.800580374788));
#38626=CARTESIAN_POINT('Ctrl Pts',(-16.2865429768018,18.4556017775032,-19.8047559387221));
#38627=CARTESIAN_POINT('Ctrl Pts',(-16.312678943375,18.3756249997159,-19.8089315026562));
#38628=CARTESIAN_POINT('Ctrl Pts',(-16.3426437089087,18.2972083995474,-19.8131070665903));
#38629=CARTESIAN_POINT('Ctrl Pts',(-16.3741219298082,18.2148311468531,-19.8174935292092));
#38630=CARTESIAN_POINT('Ctrl Pts',(-16.4098256651864,18.1341763575637,-19.8218799918281));
#38631=CARTESIAN_POINT('Ctrl Pts',(-16.4495176195312,18.0556904080171,-19.826266454447));
#38632=CARTESIAN_POINT('Ctrl Pts',(-16.4892095738761,17.9772044584704,-19.830652917066));
#38633=CARTESIAN_POINT('Ctrl Pts',(-16.5328893929524,17.9008878144519,-19.8350393796849));
#38634=CARTESIAN_POINT('Ctrl Pts',(-16.5802679097329,17.8271509896836,-19.8394258423038));
#38635=CARTESIAN_POINT('Ctrl Pts',(-16.6254664649228,17.7568069145566,-19.8436104767382));
#38636=CARTESIAN_POINT('Ctrl Pts',(-16.674199069114,17.6885486380897,-19.8477951111725));
#38637=CARTESIAN_POINT('Ctrl Pts',(-16.7262469917063,17.6227532125997,-19.8519797456069));
#38638=CARTESIAN_POINT('Ctrl Pts',(-16.778220830493,17.557051438792,-19.8561584237297));
#38639=CARTESIAN_POINT('Ctrl Pts',(-16.8335003313992,17.493805910514,-19.8603371018525));
#38640=CARTESIAN_POINT('Ctrl Pts',(-16.8918228839634,17.4333657650824,-19.8645157799753));
#38641=CARTESIAN_POINT('Ctrl Pts',(-16.9511908256749,17.3718422741984,-19.8687693578507));
#38642=CARTESIAN_POINT('Ctrl Pts',(-17.0137117247822,17.3132261339235,-19.8730229357261));
#38643=CARTESIAN_POINT('Ctrl Pts',(-17.0790648452608,17.2578513539394,-19.8772765136015));
#38644=CARTESIAN_POINT('Ctrl Pts',(-17.143150968624,17.2035501215685,-19.881447627612));
#38645=CARTESIAN_POINT('Ctrl Pts',(-17.209960109974,17.1523660019996,-19.8856187416225));
#38646=CARTESIAN_POINT('Ctrl Pts',(-17.27915312729,17.1045763538723,-19.8897898556331));
#38647=CARTESIAN_POINT('Ctrl Pts',(-17.3483229261813,17.0568027420502,-19.8939595699836));
#38648=CARTESIAN_POINT('Ctrl Pts',(-17.419874634147,17.0124216007179,-19.8981292843341));
#38649=CARTESIAN_POINT('Ctrl Pts',(-17.4934383352004,16.971668234533,-19.9022989986847));
#38650=CARTESIAN_POINT('Ctrl Pts',(-17.5669994184993,16.9309163185512,-19.9064685646565));
#38651=CARTESIAN_POINT('Ctrl Pts',(-17.642571949712,16.8937921432288,-19.9106381306283));
#38652=CARTESIAN_POINT('Ctrl Pts',(-17.7197607085089,16.8604854479081,-19.9148076966001));
#38653=CARTESIAN_POINT('Ctrl Pts',(-17.7996633275671,16.8260077308186,-19.9191238592988));
#38654=CARTESIAN_POINT('Ctrl Pts',(-17.8812974576374,16.7956211424297,-19.9234400219976));
#38655=CARTESIAN_POINT('Ctrl Pts',(-17.964203228004,16.7694814295557,-19.9277561846964));
#38656=CARTESIAN_POINT('Ctrl Pts',(-18.0444083527806,16.7441932147135,-19.9319317489096));
#38657=CARTESIAN_POINT('Ctrl Pts',(-18.1258030751548,16.7228795141883,-19.9361073131228));
#38658=CARTESIAN_POINT('Ctrl Pts',(-18.2079583914907,16.7056297227522,-19.940282877336));
#38659=CARTESIAN_POINT('Ctrl Pts',(-18.2942631757073,16.6875086857447,-19.9446693392775));
#38660=CARTESIAN_POINT('Ctrl Pts',(-18.3814068314547,16.6738729730813,-19.949055801219));
#38661=CARTESIAN_POINT('Ctrl Pts',(-18.4688855835906,16.6647646718711,-19.9534422631606));
#38662=CARTESIAN_POINT('Ctrl Pts',(-18.5563643357266,16.6556563706608,-19.9578287251021));
#38663=CARTESIAN_POINT('Ctrl Pts',(-18.6441776008593,16.6510754351691,-19.9622151870437));
#38664=CARTESIAN_POINT('Ctrl Pts',(-18.7318236815484,16.6510009250709,-19.9666016489852));
#38665=CARTESIAN_POINT('Ctrl Pts',(-18.8154370558739,16.6509298432759,-19.970786284298));
#38666=CARTESIAN_POINT('Ctrl Pts',(-18.8992095168454,16.6549593424997,-19.9749709196109));
#38667=CARTESIAN_POINT('Ctrl Pts',(-18.9827056282395,16.6631095960615,-19.9791555549237));
#38668=CARTESIAN_POINT('Ctrl Pts',(-19.0660828933656,16.6712482487571,-19.9833342339317));
#38669=CARTESIAN_POINT('Ctrl Pts',(-19.1491841362886,16.6834959609935,-19.9875129129397));
#38670=CARTESIAN_POINT('Ctrl Pts',(-19.2315736415642,16.6998209002103,-19.9916915919477));
#38671=CARTESIAN_POINT('Ctrl Pts',(-19.315439896419,16.7164384476548,-19.9959451696027));
#38672=CARTESIAN_POINT('Ctrl Pts',(-19.3985681651274,16.7372808264551,-20.0001987472577));
#38673=CARTESIAN_POINT('Ctrl Pts',(-19.4805039902948,16.7622591414211,-20.0044523249126));
#38674=CARTESIAN_POINT('Ctrl Pts',(-19.5608513518337,16.7867532097862,-20.0086234398184));
#38675=CARTESIAN_POINT('Ctrl Pts',(-19.6400516319828,16.8152241408902,-20.0127945547243));
#38676=CARTESIAN_POINT('Ctrl Pts',(-19.7176880447478,16.8475368988241,-20.0169656696301));
#38677=CARTESIAN_POINT('Ctrl Pts',(-19.7952984058594,16.8798388138978,-20.0211353848777));
#38678=CARTESIAN_POINT('Ctrl Pts',(-19.8713455174287,16.9159798188825,-20.0253051001254));
#38679=CARTESIAN_POINT('Ctrl Pts',(-19.9454312968482,16.9557762388143,-20.029474815373));
#38680=CARTESIAN_POINT('Ctrl Pts',(-20.019514439946,16.9955712426016,-20.0336443822425));
#38681=CARTESIAN_POINT('Ctrl Pts',(-20.0916359848004,17.0390211842643,-20.037813949112));
#38682=CARTESIAN_POINT('Ctrl Pts',(-20.1614224652661,17.0858964482516,-20.0419835159815));
#38683=CARTESIAN_POINT('Ctrl Pts',(-20.2336625178745,17.1344197655744,-20.0462996776219));
#38684=CARTESIAN_POINT('Ctrl Pts',(-20.3033998138015,17.1866134578917,-20.0506158392624));
#38685=CARTESIAN_POINT('Ctrl Pts',(-20.3702544757157,17.2421751498165,-20.0549320009028));
#38686=CARTESIAN_POINT('Ctrl Pts',(-20.4349313846296,17.295926950885,-20.059107566006));
#38687=CARTESIAN_POINT('Ctrl Pts',(-20.4969102614713,17.3528303456931,-20.0632831311092));
#38688=CARTESIAN_POINT('Ctrl Pts',(-20.5558837277198,17.4125729976811,-20.0674586962124));
#38689=CARTESIAN_POINT('Ctrl Pts',(-20.6178357603196,17.4753330651997,-20.0718451561215));
#38690=CARTESIAN_POINT('Ctrl Pts',(-20.6764704133144,17.5412263089033,-20.0762316160305));
#38691=CARTESIAN_POINT('Ctrl Pts',(-20.731479614623,17.6098519152915,-20.0806180759395));
#38692=CARTESIAN_POINT('Ctrl Pts',(-20.7864888159315,17.6784775216797,-20.0850045358486));
#38693=CARTESIAN_POINT('Ctrl Pts',(-20.8378722882313,17.7498349754592,-20.0893909957576));
#38694=CARTESIAN_POINT('Ctrl Pts',(-20.8853760800034,17.8234910946631,-20.0937774556667));
#38695=CARTESIAN_POINT('Ctrl Pts',(-20.9317208338504,17.8953500892083,-20.0980568909951));
#38696=CARTESIAN_POINT('Ctrl Pts',(-20.9745398785638,17.9696546343097,-20.1023363263235));
#38697=CARTESIAN_POINT('Ctrl Pts',(-21.0135728623478,18.0460332342734,-20.106615761652));
#38698=CARTESIAN_POINT('Ctrl Pts',(-21.0525424990579,18.1222878785374,-20.1108882518361));
#38699=CARTESIAN_POINT('Ctrl Pts',(-21.0877380947942,18.2006095044151,-20.1151607420202));
#38700=CARTESIAN_POINT('Ctrl Pts',(-21.118942960611,18.2805984336684,-20.1194332322043));
#38701=CARTESIAN_POINT('Ctrl Pts',(-21.1500944339135,18.3604504993293,-20.1236984120223));
#38702=CARTESIAN_POINT('Ctrl Pts',(-21.1772686129624,18.4419637894576,-20.1279635918403));
#38703=CARTESIAN_POINT('Ctrl Pts',(-21.2002957124611,18.5247161966825,-20.1322287716583));
#38704=CARTESIAN_POINT('Ctrl Pts',(-21.2232995986398,18.6073851822802,-20.136489651804));
#38705=CARTESIAN_POINT('Ctrl Pts',(-21.2421646000029,18.6912903874225,-20.1407505319496));
#38706=CARTESIAN_POINT('Ctrl Pts',(-21.2567699771926,18.7759923653821,-20.1450114120952));
#38707=CARTESIAN_POINT('Ctrl Pts',(-21.271362764314,18.8606213288853,-20.1492686192942));
#38708=CARTESIAN_POINT('Ctrl Pts',(-21.2817031594057,18.9460452737795,-20.1535258264931));
#38709=CARTESIAN_POINT('Ctrl Pts',(-21.2877212408942,19.0318134385456,-20.1577830336921));
#38710=CARTESIAN_POINT('Ctrl Pts',(-21.2919276409715,19.0917619812152,-20.1607586525376));
#38711=CARTESIAN_POINT('Ctrl Pts',(-21.2940234518455,19.1518784236118,-20.163734271383));
#38712=CARTESIAN_POINT('Ctrl Pts',(-21.293999801981,19.2120069046681,-20.1667098902285));
#38713=CARTESIAN_POINT('Origin',(-18.734,19.211,1.76670989022852));
#38714=CARTESIAN_POINT('',(-17.1744642439897,21.2411350264762,-18.8501886329194));
#38715=CARTESIAN_POINT('',(-17.1746506311395,21.2408837946619,-18.9165758925774));
#38716=CARTESIAN_POINT('',(-17.1744642439897,21.2411350264762,1.76670989022852));
#38717=CARTESIAN_POINT('',(-21.2939990581246,19.2131959965571,-19.4332901097715));
#38718=CARTESIAN_POINT('Ctrl Pts',(-17.1746506311398,21.2408837946621,-18.9165758925774));
#38719=CARTESIAN_POINT('Ctrl Pts',(-17.0075187104224,21.1151430662609,-18.9269774749334));
#38720=CARTESIAN_POINT('Ctrl Pts',(-16.2393386951681,20.375997631509,-18.97977099285));
#38721=CARTESIAN_POINT('Ctrl Pts',(-15.8675519521013,18.2379802926624,-19.074956446327));
#38722=CARTESIAN_POINT('Ctrl Pts',(-18.0006016326409,16.274093700693,-19.2021322530085));
#38723=CARTESIAN_POINT('Ctrl Pts',(-20.635918474416,16.9602241188658,-19.3215765970806));
#38724=CARTESIAN_POINT('Ctrl Pts',(-21.2889869220882,18.5174131978834,-19.3986290055925));
#38725=CARTESIAN_POINT('Ctrl Pts',(-21.2953149015357,19.2131844541912,-19.4332894785437));
#38726=CARTESIAN_POINT('Ctrl Pts',(-21.2939990581246,19.2131959965571,-19.4332901097715));
#38727=CARTESIAN_POINT('Ctrl Pts',(-21.293890587382,19.3396465586196,-19.4395926510263));
#38728=CARTESIAN_POINT('Ctrl Pts',(-21.2844099378551,19.465708927393,-19.4458951922812));
#38729=CARTESIAN_POINT('Ctrl Pts',(-21.2657470116552,19.5902849443033,-19.452197733536));
#38730=CARTESIAN_POINT('Ctrl Pts',(-21.2615163488398,19.618524841776,-19.4536264444811));
#38731=CARTESIAN_POINT('Ctrl Pts',(-21.2568139996567,19.6466884925667,-19.4550551554262));
#38732=CARTESIAN_POINT('Ctrl Pts',(-21.2516424693627,19.6747632978808,-19.4564838663713));
#38733=CARTESIAN_POINT('Ctrl Pts',(-21.2364952751686,19.7569932189831,-19.4606685004935));
#38734=CARTESIAN_POINT('Ctrl Pts',(-21.2172870302474,19.8386332916553,-19.4648531346158));
#38735=CARTESIAN_POINT('Ctrl Pts',(-21.1940771445785,19.9192516803528,-19.469037768738));
#38736=CARTESIAN_POINT('Ctrl Pts',(-21.1709002953099,19.9997553187496,-19.4732164465514));
#38737=CARTESIAN_POINT('Ctrl Pts',(-21.1437332452095,20.0792397234556,-19.4773951243647));
#38738=CARTESIAN_POINT('Ctrl Pts',(-21.1126865924437,20.1572822490824,-19.4815738021781));
#38739=CARTESIAN_POINT('Ctrl Pts',(-21.0810834481907,20.2367236373009,-19.4858273801312));
#38740=CARTESIAN_POINT('Ctrl Pts',(-21.0454603361894,20.3146704722382,-19.4900809580843));
#38741=CARTESIAN_POINT('Ctrl Pts',(-21.0059873753743,20.3906920641166,-19.4943345360374));
#38742=CARTESIAN_POINT('Ctrl Pts',(-20.9672796780334,20.4652398231152,-19.4985056497473));
#38743=CARTESIAN_POINT('Ctrl Pts',(-20.9248702957982,20.5379358953033,-19.5026767634572));
#38744=CARTESIAN_POINT('Ctrl Pts',(-20.8789678616489,20.6083950309391,-19.506847877167));
#38745=CARTESIAN_POINT('Ctrl Pts',(-20.8330808304891,20.6788305233554,-19.5110175912208));
#38746=CARTESIAN_POINT('Ctrl Pts',(-20.7837033261796,20.7470301848417,-19.5151873052746));
#38747=CARTESIAN_POINT('Ctrl Pts',(-20.7310884045781,20.8126360086797,-19.5193570193284));
#38748=CARTESIAN_POINT('Ctrl Pts',(-20.6784753552182,20.8782394980099,-19.5235265850078));
#38749=CARTESIAN_POINT('Ctrl Pts',(-20.6226254060923,20.9412489748611,-19.5276961506871));
#38750=CARTESIAN_POINT('Ctrl Pts',(-20.5638323063888,21.0013389987641,-19.5318657163664));
#38751=CARTESIAN_POINT('Ctrl Pts',(-20.502972105477,21.0635417223146,-19.5361818794236));
#38752=CARTESIAN_POINT('Ctrl Pts',(-20.4389583088965,21.122615499409,-19.5404980424808));
#38753=CARTESIAN_POINT('Ctrl Pts',(-20.3721573780251,21.1782418267264,-19.544814205538));
#38754=CARTESIAN_POINT('Ctrl Pts',(-20.3075324892011,21.2320561249956,-19.5489897694722));
#38755=CARTESIAN_POINT('Ctrl Pts',(-20.2402996648593,21.2826438810762,-19.5531653334064));
#38756=CARTESIAN_POINT('Ctrl Pts',(-20.1708219662268,21.329759693162,-19.5573408973406));
#38757=CARTESIAN_POINT('Ctrl Pts',(-20.0978350996175,21.3792552228008,-19.5617273599593));
#38758=CARTESIAN_POINT('Ctrl Pts',(-20.0223711202591,21.4249185513468,-19.566113822578));
#38759=CARTESIAN_POINT('Ctrl Pts',(-19.9448802161397,21.4665196966911,-19.5705002851967));
#38760=CARTESIAN_POINT('Ctrl Pts',(-19.8673893120203,21.5081208420354,-19.5748867478154));
#38761=CARTESIAN_POINT('Ctrl Pts',(-19.7878720403016,21.5456596252664,-19.579273210434));
#38762=CARTESIAN_POINT('Ctrl Pts',(-19.7068005673304,21.5789651720837,-19.5836596730527));
#38763=CARTESIAN_POINT('Ctrl Pts',(-19.629459322931,21.6107382772446,-19.5878443074871));
#38764=CARTESIAN_POINT('Ctrl Pts',(-19.5504158778411,21.6387774071505,-19.5920289419215));
#38765=CARTESIAN_POINT('Ctrl Pts',(-19.4700654949587,21.6628987717953,-19.5962135763559));
#38766=CARTESIAN_POINT('Ctrl Pts',(-19.3898294809474,21.6869858026491,-19.6003922544787));
#38767=CARTESIAN_POINT('Ctrl Pts',(-19.3082906610537,21.7071660136986,-19.6045709326015));
#38768=CARTESIAN_POINT('Ctrl Pts',(-19.2258642779018,21.7233036305598,-19.6087496107243));
#38769=CARTESIAN_POINT('Ctrl Pts',(-19.1419604620487,21.7397305024139,-19.6130031885997));
#38770=CARTESIAN_POINT('Ctrl Pts',(-19.0571373968166,21.7519682444677,-19.6172567664751));
#38771=CARTESIAN_POINT('Ctrl Pts',(-18.9718493062277,21.7599267756307,-19.6215103443505));
#38772=CARTESIAN_POINT('Ctrl Pts',(-18.8882146908505,21.7677310152166,-19.6256814583611));
#38773=CARTESIAN_POINT('Ctrl Pts',(-18.8041333991885,21.7714204401683,-19.6298525723716));
#38774=CARTESIAN_POINT('Ctrl Pts',(-18.7200422944287,21.7709619494155,-19.6340236863821));
#38775=CARTESIAN_POINT('Ctrl Pts',(-18.6359794072993,21.7705036125139,-19.6381934007327));
#38776=CARTESIAN_POINT('Ctrl Pts',(-18.551907173255,21.7659001267009,-19.6423631150832));
#38777=CARTESIAN_POINT('Ctrl Pts',(-18.4682635936743,21.7571704896477,-19.6465328294338));
#38778=CARTESIAN_POINT('Ctrl Pts',(-18.3846229905396,21.7484411632376,-19.6507023954056));
#38779=CARTESIAN_POINT('Ctrl Pts',(-18.3014114689995,21.7355860261208,-19.6548719613774));
#38780=CARTESIAN_POINT('Ctrl Pts',(-18.2190616739018,21.7186759201131,-19.6590415273492));
#38781=CARTESIAN_POINT('Ctrl Pts',(-18.1338165629591,21.7011712759185,-19.663357690048));
#38782=CARTESIAN_POINT('Ctrl Pts',(-18.0494954191338,21.679321318249,-19.6676738527467));
#38783=CARTESIAN_POINT('Ctrl Pts',(-17.966564411757,21.6532617832448,-19.6719900154455));
#38784=CARTESIAN_POINT('Ctrl Pts',(-17.8863348720621,21.6280511344877,-19.6761655796587));
#38785=CARTESIAN_POINT('Ctrl Pts',(-17.8074067178008,21.5989011580654,-19.6803411438719));
#38786=CARTESIAN_POINT('Ctrl Pts',(-17.7301828112741,21.5659842996543,-19.6845167080851));
#38787=CARTESIAN_POINT('Ctrl Pts',(-17.6490585105433,21.5314048897156,-19.6889031700266));
#38788=CARTESIAN_POINT('Ctrl Pts',(-17.5698156696645,21.4926683234483,-19.6932896319682));
#38789=CARTESIAN_POINT('Ctrl Pts',(-17.492891345209,21.4500286525641,-19.6976760939097));
#38790=CARTESIAN_POINT('Ctrl Pts',(-17.4159670207535,21.4073889816798,-19.7020625558512));
#38791=CARTESIAN_POINT('Ctrl Pts',(-17.341361664738,21.3608465778214,-19.7064490177927));
#38792=CARTESIAN_POINT('Ctrl Pts',(-17.2694745299336,21.3107059669218,-19.7108354797342));
#38793=CARTESIAN_POINT('Ctrl Pts',(-17.2373037292364,21.2882671313154,-19.7127985012577));
#38794=CARTESIAN_POINT('Ctrl Pts',(-17.2056207285748,21.2650692235164,-19.7147615227813));
#38795=CARTESIAN_POINT('Ctrl Pts',(-17.1744642439897,21.2411350264762,-19.7167245443048));
#38796=CARTESIAN_POINT('',(-21.2939989850552,19.2087204131754,-19.3667098901939));
#38797=CARTESIAN_POINT('Ctrl Pts',(-21.2939989850559,19.2087204138716,-19.3667098902285));
#38798=CARTESIAN_POINT('Ctrl Pts',(-21.294073180434,19.292042596975,-19.3708480242597));
#38799=CARTESIAN_POINT('Ctrl Pts',(-21.2900751830218,19.3754486069202,-19.374986158291));
#38800=CARTESIAN_POINT('Ctrl Pts',(-21.2820071809338,19.4585063754929,-19.3791242923222));
#38801=CARTESIAN_POINT('Ctrl Pts',(-21.2739428344705,19.541526510458,-19.3832605513583));
#38802=CARTESIAN_POINT('Ctrl Pts',(-21.2618121886757,19.6241982519104,-19.3873968103944));
#38803=CARTESIAN_POINT('Ctrl Pts',(-21.2456694473256,19.7060925038528,-19.3915330694305));
#38804=CARTESIAN_POINT('Ctrl Pts',(-21.2295289836483,19.7879752008609,-19.3956687448579));
#38805=CARTESIAN_POINT('Ctrl Pts',(-21.2093776397595,19.8690801670299,-19.3998044202852));
#38806=CARTESIAN_POINT('Ctrl Pts',(-21.1853208566118,19.9489878440326,-19.4039400957126));
#38807=CARTESIAN_POINT('Ctrl Pts',(-21.1612599617805,20.0289091785175,-19.4080764779921));
#38808=CARTESIAN_POINT('Ctrl Pts',(-21.1332924395122,20.1076323699233,-19.4122128602716));
#38809=CARTESIAN_POINT('Ctrl Pts',(-21.1015733410929,20.1847538059213,-19.4163492425511));
#38810=CARTESIAN_POINT('Ctrl Pts',(-21.0698191717518,20.2619605129384,-19.420490198313));
#38811=CARTESIAN_POINT('Ctrl Pts',(-21.0343053289548,20.3375614976483,-19.4246311540749));
#38812=CARTESIAN_POINT('Ctrl Pts',(-20.9952344193577,20.4111745292715,-19.4287721098369));
#38813=CARTESIAN_POINT('Ctrl Pts',(-20.956138222721,20.4848352039023,-19.4329157456621));
#38814=CARTESIAN_POINT('Ctrl Pts',(-20.9134806196,20.5565049647657,-19.4370593814874));
#38815=CARTESIAN_POINT('Ctrl Pts',(-20.8675081508492,20.6258296612172,-19.4412030173127));
#38816=CARTESIAN_POINT('Ctrl Pts',(-20.8214607545843,20.6952673454484,-19.4453534065784));
#38817=CARTESIAN_POINT('Ctrl Pts',(-20.7720879921639,20.7623519651645,-19.4495037958442));
#38818=CARTESIAN_POINT('Ctrl Pts',(-20.7196769297106,20.8267620897939,-19.4536541851099));
#38819=CARTESIAN_POINT('Ctrl Pts',(-20.701811538935,20.8487176082006,-19.4550689308264));
#38820=CARTESIAN_POINT('Ctrl Pts',(-20.6835934338612,20.8703626873999,-19.456483676543));
#38821=CARTESIAN_POINT('Ctrl Pts',(-20.665034920053,20.8916856153177,-19.4578984222595));
#38822=CARTESIAN_POINT('Ctrl Pts',(-20.6101412425939,20.9547560712659,-19.4620830566462));
#38823=CARTESIAN_POINT('Ctrl Pts',(-20.5520521994161,21.0152517076034,-19.466267691033));
#38824=CARTESIAN_POINT('Ctrl Pts',(-20.4910387353968,21.0728310563301,-19.4704523254197));
#38825=CARTESIAN_POINT('Ctrl Pts',(-20.4301121164969,21.1303284479757,-19.474631003497));
#38826=CARTESIAN_POINT('Ctrl Pts',(-20.3662696766025,21.1849174841126,-19.4788096815743));
#38827=CARTESIAN_POINT('Ctrl Pts',(-20.2998217436364,21.2362906623878,-19.4829883596516));
#38828=CARTESIAN_POINT('Ctrl Pts',(-20.2321827790938,21.2885846680655,-19.4872419375387));
#38829=CARTESIAN_POINT('Ctrl Pts',(-20.161844312329,21.3375460297091,-19.4914955154257));
#38830=CARTESIAN_POINT('Ctrl Pts',(-20.0891719990913,21.3828906171534,-19.4957490933128));
#38831=CARTESIAN_POINT('Ctrl Pts',(-20.0179085806091,21.4273561111906,-19.4999202072832));
#38832=CARTESIAN_POINT('Ctrl Pts',(-19.9444014087256,21.4683435613089,-19.5040913212537));
#38833=CARTESIAN_POINT('Ctrl Pts',(-19.8690261614781,21.5056275542581,-19.5082624352241));
#38834=CARTESIAN_POINT('Ctrl Pts',(-19.793676207128,21.5428990362007,-19.5124321495367));
#38835=CARTESIAN_POINT('Ctrl Pts',(-19.7164598343519,21.5764693252628,-19.5166018638493));
#38836=CARTESIAN_POINT('Ctrl Pts',(-19.6377770918877,21.6061590694939,-19.5207715781619));
#38837=CARTESIAN_POINT('Ctrl Pts',(-19.5590971492983,21.6358477572345,-19.5249411440979));
#38838=CARTESIAN_POINT('Ctrl Pts',(-19.4789513714795,21.6616560130841,-19.5291107100339));
#38839=CARTESIAN_POINT('Ctrl Pts',(-19.3977582580605,21.6834532300645,-19.5332802759699));
#38840=CARTESIAN_POINT('Ctrl Pts',(-19.313710494605,21.706016810393,-19.5375964387175));
#38841=CARTESIAN_POINT('Ctrl Pts',(-19.2285408859855,21.7242819108903,-19.541912601465));
#38842=CARTESIAN_POINT('Ctrl Pts',(-19.1427269885521,21.7381609067942,-19.5462287642126));
#38843=CARTESIAN_POINT('Ctrl Pts',(-19.0597084701407,21.7515877958115,-19.5504043283956));
#38844=CARTESIAN_POINT('Ctrl Pts',(-18.9760874671013,21.7609099414407,-19.5545798925786));
#38845=CARTESIAN_POINT('Ctrl Pts',(-18.8923014001317,21.7661009112589,-19.5587554567616));
#38846=CARTESIAN_POINT('Ctrl Pts',(-18.8042834975712,21.7715540646552,-19.5631419187915));
#38847=CARTESIAN_POINT('Ctrl Pts',(-18.716084001952,21.7724477372194,-19.5675283808214));
#38848=CARTESIAN_POINT('Ctrl Pts',(-18.6282074804569,21.7688131172564,-19.5719148428513));
#38849=CARTESIAN_POINT('Ctrl Pts',(-18.5403309589617,21.7651784972933,-19.5763013048811));
#38850=CARTESIAN_POINT('Ctrl Pts',(-18.4527779822413,21.7570157144011,-19.580687766911));
#38851=CARTESIAN_POINT('Ctrl Pts',(-18.3660419494175,21.7444180217665,-19.5850742289409));
#38852=CARTESIAN_POINT('Ctrl Pts',(-18.2832980106589,21.7324001478343,-19.5892588006091));
#38853=CARTESIAN_POINT('Ctrl Pts',(-18.2009894838862,21.7163018984357,-19.5934433722773));
#38854=CARTESIAN_POINT('Ctrl Pts',(-18.1195501274672,21.6961662628775,-19.5976279439455));
#38855=CARTESIAN_POINT('Ctrl Pts',(-18.0344368609572,21.6751222641161,-19.6020012909277));
#38856=CARTESIAN_POINT('Ctrl Pts',(-17.9502735392786,21.6496679882501,-19.6063746379099));
#38857=CARTESIAN_POINT('Ctrl Pts',(-17.8675488737407,21.6199131254165,-19.610747984892));
#38858=CARTESIAN_POINT('Ctrl Pts',(-17.7886022149566,21.5915171568379,-19.6149216026359));
#38859=CARTESIAN_POINT('Ctrl Pts',(-17.7109661880779,21.5592049570797,-19.6190952203798));
#38860=CARTESIAN_POINT('Ctrl Pts',(-17.6350528734777,21.5231235289466,-19.6232688381237));
#38861=CARTESIAN_POINT('Ctrl Pts',(-17.5591911030165,21.4870665996271,-19.6274396220362));
#38862=CARTESIAN_POINT('Ctrl Pts',(-17.4850501355258,21.447245722735,-19.6316104059488));
#38863=CARTESIAN_POINT('Ctrl Pts',(-17.413022153431,21.4038560210087,-19.6357811898613));
#38864=CARTESIAN_POINT('Ctrl Pts',(-17.3410199038859,21.3604818205865,-19.6399504837292));
#38865=CARTESIAN_POINT('Ctrl Pts',(-17.2711295331142,21.3135415662574,-19.6441197775971));
#38866=CARTESIAN_POINT('Ctrl Pts',(-17.203717503422,21.2632756833981,-19.6482890714651));
#38867=CARTESIAN_POINT('Ctrl Pts',(-17.1939136908581,21.2559654555921,-19.6488954168873));
#38868=CARTESIAN_POINT('Ctrl Pts',(-17.1841622460799,21.2485849649405,-19.6495017623095));
#38869=CARTESIAN_POINT('Ctrl Pts',(-17.1744642439897,21.2411350264762,-19.6501081077317));
#38870=CARTESIAN_POINT('Ctrl Pts',(-17.1744642439897,21.2411350264762,-18.8501886329194));
#38871=CARTESIAN_POINT('Ctrl Pts',(-17.1079120298185,21.1900100735602,-18.8543616881065));
#38872=CARTESIAN_POINT('Ctrl Pts',(-17.0438081666524,21.1355566463855,-18.8585347432936));
#38873=CARTESIAN_POINT('Ctrl Pts',(-16.9824993407833,21.0780418958244,-18.8627077984807));
#38874=CARTESIAN_POINT('Ctrl Pts',(-16.9212253091811,21.020559786299,-18.8668784853563));
#38875=CARTESIAN_POINT('Ctrl Pts',(-16.8627435002704,20.9600201168211,-18.8710491722319));
#38876=CARTESIAN_POINT('Ctrl Pts',(-16.8073668119571,20.8967296813936,-18.8752198591075));
#38877=CARTESIAN_POINT('Ctrl Pts',(-16.7520049394097,20.833456179017,-18.879389430136));
#38878=CARTESIAN_POINT('Ctrl Pts',(-16.6997468400686,20.7674337185571,-18.8835590011644));
#38879=CARTESIAN_POINT('Ctrl Pts',(-16.6508669315501,20.6990042402932,-18.8877285721929));
#38880=CARTESIAN_POINT('Ctrl Pts',(-16.6019854379048,20.6305725429294,-18.8918982784364));
#38881=CARTESIAN_POINT('Ctrl Pts',(-16.5564826189569,20.559734047872,-18.8960679846799));
#38882=CARTESIAN_POINT('Ctrl Pts',(-16.5145903334575,20.4868607808291,-18.9002376909234));
#38883=CARTESIAN_POINT('Ctrl Pts',(-16.4726553116461,20.4139131723019,-18.9044116508825));
#38884=CARTESIAN_POINT('Ctrl Pts',(-16.4343384099249,20.3389270454576,-18.9085856108416));
#38885=CARTESIAN_POINT('Ctrl Pts',(-16.3998258981524,20.262299796568,-18.9127595708007));
#38886=CARTESIAN_POINT('Ctrl Pts',(-16.3652960666188,20.185634093055,-18.9169356254201));
#38887=CARTESIAN_POINT('Ctrl Pts',(-16.3345745959917,20.1073260557597,-18.9211116800395));
#38888=CARTESIAN_POINT('Ctrl Pts',(-16.3077989545311,20.0277915811058,-18.9252877346589));
#38889=CARTESIAN_POINT('Ctrl Pts',(-16.2809755043854,19.9481150953389,-18.9294712457451));
#38890=CARTESIAN_POINT('Ctrl Pts',(-16.2581120855318,19.8672082404936,-18.9336547568312));
#38891=CARTESIAN_POINT('Ctrl Pts',(-16.239295758604,19.7855004333862,-18.9378382679174));
#38892=CARTESIAN_POINT('Ctrl Pts',(-16.2222689392233,19.7115633637894,-18.9416239104561));
#38893=CARTESIAN_POINT('Ctrl Pts',(-16.2085553993355,19.6369708281993,-18.9454095529949));
#38894=CARTESIAN_POINT('Ctrl Pts',(-16.1981829862585,19.5620442604845,-18.9491951955337));
#38895=CARTESIAN_POINT('Ctrl Pts',(-16.1867173615958,19.4792207269146,-18.9533798299225));
#38896=CARTESIAN_POINT('Ctrl Pts',(-16.1792923755172,19.3956807451282,-18.9575644643113));
#38897=CARTESIAN_POINT('Ctrl Pts',(-16.1759873564286,19.3118529391175,-18.9617490987001));
#38898=CARTESIAN_POINT('Ctrl Pts',(-16.1726870416255,19.2281444516126,-18.9659277767798));
#38899=CARTESIAN_POINT('Ctrl Pts',(-16.173495063509,19.1441494093852,-18.9701064548596));
#38900=CARTESIAN_POINT('Ctrl Pts',(-16.1784392678899,19.0603038006558,-18.9742851329393));
#38901=CARTESIAN_POINT('Ctrl Pts',(-16.1834720935873,18.9749553195411,-18.9785387108258));
#38902=CARTESIAN_POINT('Ctrl Pts',(-16.1927909085457,18.8897621593934,-18.9827922887123));
#38903=CARTESIAN_POINT('Ctrl Pts',(-16.2063695825696,18.8051866526586,-18.9870458665988));
#38904=CARTESIAN_POINT('Ctrl Pts',(-16.2196850074843,18.7222508072609,-18.9912169805725));
#38905=CARTESIAN_POINT('Ctrl Pts',(-16.2370965177706,18.6399093552907,-18.9953880945463));
#38906=CARTESIAN_POINT('Ctrl Pts',(-16.2585271389987,18.5585935971759,-18.9995592085201));
#38907=CARTESIAN_POINT('Ctrl Pts',(-16.279950568975,18.4773051253486,-19.0037289228363));
#38908=CARTESIAN_POINT('Ctrl Pts',(-16.3053903143098,18.3970421083,-19.0078986371526));
#38909=CARTESIAN_POINT('Ctrl Pts',(-16.3347186663499,18.3182239463347,-19.0120683514688));
#38910=CARTESIAN_POINT('Ctrl Pts',(-16.3640459747616,18.2394085890572,-19.0162379174088));
#38911=CARTESIAN_POINT('Ctrl Pts',(-16.3972614535261,18.1620384154931,-19.0204074833487));
#38912=CARTESIAN_POINT('Ctrl Pts',(-16.4341885271975,18.0865147001558,-19.0245770492886));
#38913=CARTESIAN_POINT('Ctrl Pts',(-16.4724139113061,18.0083356639891,-19.0288932120325));
#38914=CARTESIAN_POINT('Ctrl Pts',(-16.5146165141609,17.9321358186698,-19.0332093747764));
#38915=CARTESIAN_POINT('Ctrl Pts',(-16.5605485527344,17.8583327066942,-19.0375255375203));
#38916=CARTESIAN_POINT('Ctrl Pts',(-16.6049843598894,17.7869337234784,-19.041701101708));
#38917=CARTESIAN_POINT('Ctrl Pts',(-16.6529100541822,17.7177780846058,-19.0458766658957));
#38918=CARTESIAN_POINT('Ctrl Pts',(-16.7040581042278,17.651212867155,-19.0500522300834));
#38919=CARTESIAN_POINT('Ctrl Pts',(-16.7577895208549,17.5812855985979,-19.0544386921054));
#38920=CARTESIAN_POINT('Ctrl Pts',(-16.8150769912951,17.5142177570115,-19.0588251541273));
#38921=CARTESIAN_POINT('Ctrl Pts',(-16.8755654265148,17.4503691653061,-19.0632116161493));
#38922=CARTESIAN_POINT('Ctrl Pts',(-16.9360538617345,17.3865205736007,-19.0675980781712));
#38923=CARTESIAN_POINT('Ctrl Pts',(-16.9997427890408,17.3258915767388,-19.0719845401932));
#38924=CARTESIAN_POINT('Ctrl Pts',(-17.0662376770542,17.2687927931957,-19.0763710022152));
#38925=CARTESIAN_POINT('Ctrl Pts',(-17.1296730365262,17.2143212094742,-19.0805556366057));
#38926=CARTESIAN_POINT('Ctrl Pts',(-17.1958979365981,17.1628593635266,-19.0847402709962));
#38927=CARTESIAN_POINT('Ctrl Pts',(-17.2645949112854,17.1147059640261,-19.0889249053867));
#38928=CARTESIAN_POINT('Ctrl Pts',(-17.3331941043313,17.0666211049302,-19.093103583468));
#38929=CARTESIAN_POINT('Ctrl Pts',(-17.4042580092797,17.0218356001939,-19.0972822615493));
#38930=CARTESIAN_POINT('Ctrl Pts',(-17.4774351014431,16.9806088558922,-19.1014609396307));
#38931=CARTESIAN_POINT('Ctrl Pts',(-17.5519238404496,16.9386431517955,-19.1057145175168));
#38932=CARTESIAN_POINT('Ctrl Pts',(-17.6286019037991,16.9003653586862,-19.1099680954028));
#38933=CARTESIAN_POINT('Ctrl Pts',(-17.7070663992917,16.8660037569889,-19.1142216732889));
#38934=CARTESIAN_POINT('Ctrl Pts',(-17.7840097073668,16.8323083220186,-19.1183927872642));
#38935=CARTESIAN_POINT('Ctrl Pts',(-17.862670357959,16.8023787805161,-19.1225639012394));
#38936=CARTESIAN_POINT('Ctrl Pts',(-17.942644030864,16.7763838639094,-19.1267350152146));
#38937=CARTESIAN_POINT('Ctrl Pts',(-18.0225908678302,16.7503976701481,-19.1309047295323));
#38938=CARTESIAN_POINT('Ctrl Pts',(-18.1038494149387,16.7283436212316,-19.1350744438499));
#38939=CARTESIAN_POINT('Ctrl Pts',(-18.185997896633,16.7103413478235,-19.1392441581675));
#38940=CARTESIAN_POINT('Ctrl Pts',(-18.2681434551313,16.6923397150136,-19.1434137241088));
#38941=CARTESIAN_POINT('Ctrl Pts',(-18.3511784357002,16.6783896686898,-19.1475832900501));
#38942=CARTESIAN_POINT('Ctrl Pts',(-18.4346698530371,16.6685599391295,-19.1517528559914));
#38943=CARTESIAN_POINT('Ctrl Pts',(-18.5210967257309,16.6583846083899,-19.1560690187335));
#38944=CARTESIAN_POINT('Ctrl Pts',(-18.6080122052096,16.6526247876704,-19.1603851814756));
#38945=CARTESIAN_POINT('Ctrl Pts',(-18.6949310840593,16.6512981384921,-19.1647013442177));
#38946=CARTESIAN_POINT('Ctrl Pts',(-18.7790185894541,16.650014704773,-19.1688769084065));
#38947=CARTESIAN_POINT('Ctrl Pts',(-18.8631088069912,16.652879993597,-19.1730524725954));
#38948=CARTESIAN_POINT('Ctrl Pts',(-18.946765090109,16.6598569196474,-19.1772280367842));
#38949=CARTESIAN_POINT('Ctrl Pts',(-19.0346466533962,16.6671862336619,-19.181614498803));
#38950=CARTESIAN_POINT('Ctrl Pts',(-19.1220487156005,16.6790533797552,-19.1860009608217));
#38951=CARTESIAN_POINT('Ctrl Pts',(-19.2084765196395,16.6953545495617,-19.1903874228404));
#38952=CARTESIAN_POINT('Ctrl Pts',(-19.2949043236785,16.7116557193682,-19.1947738848591));
#38953=CARTESIAN_POINT('Ctrl Pts',(-19.3803573236336,16.7323907021497,-19.1991603468778));
#38954=CARTESIAN_POINT('Ctrl Pts',(-19.4643607861717,16.7573958913422,-19.2035468088965));
#38955=CARTESIAN_POINT('Ctrl Pts',(-19.5444991251657,16.7812505547997,-19.2077314433106));
#38956=CARTESIAN_POINT('Ctrl Pts',(-19.6236166763879,16.8090798944626,-19.2119160777247));
#38957=CARTESIAN_POINT('Ctrl Pts',(-19.7012904347963,16.8407786570129,-19.2161007121388));
#38958=CARTESIAN_POINT('Ctrl Pts',(-19.7788536342255,16.872432300299,-19.2202793902439));
#38959=CARTESIAN_POINT('Ctrl Pts',(-19.8549767005509,16.907944254222,-19.2244580683489));
#38960=CARTESIAN_POINT('Ctrl Pts',(-19.9292512406659,16.9471593537339,-19.228636746454));
#38961=CARTESIAN_POINT('Ctrl Pts',(-20.0048570980567,16.98707735547,-19.2328903243342));
#38962=CARTESIAN_POINT('Ctrl Pts',(-20.0785470456703,17.0308324287623,-19.2371439022144));
#38963=CARTESIAN_POINT('Ctrl Pts',(-20.1499110578951,17.0782093688947,-19.2413974800945));
#38964=CARTESIAN_POINT('Ctrl Pts',(-20.2198915399285,17.1246678148869,-19.2455685940936));
#38965=CARTESIAN_POINT('Ctrl Pts',(-20.287635066423,17.1746086809011,-19.2497397080927));
#38966=CARTESIAN_POINT('Ctrl Pts',(-20.3527809100897,17.2277833287487,-19.2539108220917));
#38967=CARTESIAN_POINT('Ctrl Pts',(-20.4179048934388,17.2809401333292,-19.2580805364332));
#38968=CARTESIAN_POINT('Ctrl Pts',(-20.4804325690374,17.3373282740108,-19.2622502507746));
#38969=CARTESIAN_POINT('Ctrl Pts',(-20.5400350473177,17.3966578581039,-19.2664199651161));
#38970=CARTESIAN_POINT('Ctrl Pts',(-20.5996354046851,17.4559853309948,-19.2705895310811));
#38971=CARTESIAN_POINT('Ctrl Pts',(-20.6563104462573,17.5182537140387,-19.2747590970462));
#38972=CARTESIAN_POINT('Ctrl Pts',(-20.7097680140133,17.5831361375097,-19.2789286630112));
#38973=CARTESIAN_POINT('Ctrl Pts',(-20.7651050833052,17.6502997462213,-19.2832448257251));
#38974=CARTESIAN_POINT('Ctrl Pts',(-20.8169938810692,17.7202642276974,-19.287560988439));
#38975=CARTESIAN_POINT('Ctrl Pts',(-20.8651569231979,17.7926311591459,-19.2918771511529));
#38976=CARTESIAN_POINT('Ctrl Pts',(-20.9117510597951,17.8626407461655,-19.2960527153652));
#38977=CARTESIAN_POINT('Ctrl Pts',(-20.9548582452775,17.9348982385164,-19.3002282795775));
#38978=CARTESIAN_POINT('Ctrl Pts',(-20.9942733140221,18.0090164119592,-19.3044038437898));
#38979=CARTESIAN_POINT('Ctrl Pts',(-21.0356791435328,18.0868781169101,-19.3087903057545));
#38980=CARTESIAN_POINT('Ctrl Pts',(-21.0730098296529,18.1667928797187,-19.3131767677192));
#38981=CARTESIAN_POINT('Ctrl Pts',(-21.1060848561709,18.2482884984978,-19.3175632296839));
#38982=CARTESIAN_POINT('Ctrl Pts',(-21.1391598826889,18.329784117277,-19.3219496916486));
#38983=CARTESIAN_POINT('Ctrl Pts',(-21.1679791313067,18.4128600189272,-19.3263361536133));
#38984=CARTESIAN_POINT('Ctrl Pts',(-21.1924232051052,18.4970284707355,-19.330722615578));
#38985=CARTESIAN_POINT('Ctrl Pts',(-21.2214742546483,18.5970601546363,-19.3359357942367));
#38986=CARTESIAN_POINT('Ctrl Pts',(-21.2444357643533,18.6989346521836,-19.3411489728953));
#38987=CARTESIAN_POINT('Ctrl Pts',(-21.2611151500594,18.8019901977457,-19.3463621515539));
#38988=CARTESIAN_POINT('Ctrl Pts',(-21.2775287210165,18.9034033756297,-19.3514922492285));
#38989=CARTESIAN_POINT('Ctrl Pts',(-21.2878587863005,19.0059603454814,-19.3566223469032));
#38990=CARTESIAN_POINT('Ctrl Pts',(-21.2919675308107,19.1090092586637,-19.3617524445778));
#38991=CARTESIAN_POINT('Ctrl Pts',(-21.2932910194166,19.1422028685647,-19.3634049264499));
#38992=CARTESIAN_POINT('Ctrl Pts',(-21.2939693565913,19.1754473495009,-19.3650574083219));
#38993=CARTESIAN_POINT('Ctrl Pts',(-21.2939989850552,19.2087204131754,-19.3667098901939));
#38994=CARTESIAN_POINT('Origin',(-18.734,19.211,1.76670989022852));
#38995=CARTESIAN_POINT('',(-17.1744642439897,21.2411350264762,-18.0500683119931));
#38996=CARTESIAN_POINT('',(-17.1744642439897,21.2411350264762,-18.1167065484839));
#38997=CARTESIAN_POINT('',(-17.1744642439897,21.2411350264762,1.76670989022852));
#38998=CARTESIAN_POINT('',(-21.2936055415609,19.2113823947434,-18.6332901348857));
#38999=CARTESIAN_POINT('Ctrl Pts',(-17.1744642439897,21.2411350264762,-18.1167065484839));
#39000=CARTESIAN_POINT('Ctrl Pts',(-17.1077795034155,21.1899082676894,-18.1208760279071));
#39001=CARTESIAN_POINT('Ctrl Pts',(-17.0436130429836,21.1353860024748,-18.1250455073302));
#39002=CARTESIAN_POINT('Ctrl Pts',(-16.9822981323806,21.0778531187478,-18.1292149867534));
#39003=CARTESIAN_POINT('Ctrl Pts',(-16.9209724759196,21.0203101519891,-18.1333851969064));
#39004=CARTESIAN_POINT('Ctrl Pts',(-16.8624996961633,20.9597558347282,-18.1375554070594));
#39005=CARTESIAN_POINT('Ctrl Pts',(-16.807176747738,20.8965124308478,-18.1417256172124));
#39006=CARTESIAN_POINT('Ctrl Pts',(-16.7517926921237,20.8331991712069,-18.145900433588));
#39007=CARTESIAN_POINT('Ctrl Pts',(-16.6995657146274,20.7671912439353,-18.1500752499637));
#39008=CARTESIAN_POINT('Ctrl Pts',(-16.6507525780277,20.6988441379545,-18.1542500663394));
#39009=CARTESIAN_POINT('Ctrl Pts',(-16.6019086931009,20.6304539788262,-18.1584275125116));
#39010=CARTESIAN_POINT('Ctrl Pts',(-16.5564831775601,20.559722095032,-18.1626049586839));
#39011=CARTESIAN_POINT('Ctrl Pts',(-16.5146882374202,20.4870310734755,-18.1667824048561));
#39012=CARTESIAN_POINT('Ctrl Pts',(-16.4728247886002,20.4142208995544,-18.1709666985396));
#39013=CARTESIAN_POINT('Ctrl Pts',(-16.4346040018293,20.3394455874191,-18.1751509922232));
#39014=CARTESIAN_POINT('Ctrl Pts',(-16.4001909244614,20.2631098796863,-18.1793352859067));
#39015=CARTESIAN_POINT('Ctrl Pts',(-16.385413108711,20.2303294627539,-18.1811321237901));
#39016=CARTESIAN_POINT('Ctrl Pts',(-16.371336836165,20.1972615163169,-18.1829289616735));
#39017=CARTESIAN_POINT('Ctrl Pts',(-16.3579723492966,20.1639389293617,-18.184725799557));
#39018=CARTESIAN_POINT('Ctrl Pts',(-16.3268479546498,20.0863343526005,-18.1889104339505));
#39019=CARTESIAN_POINT('Ctrl Pts',(-16.2994716572956,20.00705890033,-18.193095068344));
#39020=CARTESIAN_POINT('Ctrl Pts',(-16.2760239311543,19.926509360513,-18.1972797027374));
#39021=CARTESIAN_POINT('Ctrl Pts',(-16.252609579949,19.846074472996,-18.2014583808218));
#39022=CARTESIAN_POINT('Ctrl Pts',(-16.2331128202905,19.7643695380471,-18.2056370589062));
#39023=CARTESIAN_POINT('Ctrl Pts',(-16.217665944864,19.681810920607,-18.2098157369906));
#39024=CARTESIAN_POINT('Ctrl Pts',(-16.2019421952991,19.5977724992941,-18.2140693148759));
#39025=CARTESIAN_POINT('Ctrl Pts',(-16.190415125853,19.512849937439,-18.2183228927612));
#39026=CARTESIAN_POINT('Ctrl Pts',(-16.1831710111198,19.4274981974256,-18.2225764706466));
#39027=CARTESIAN_POINT('Ctrl Pts',(-16.1760673376856,19.3438011674318,-18.226747584625));
#39028=CARTESIAN_POINT('Ctrl Pts',(-16.1730820747445,19.2596919311862,-18.2309186986033));
#39029=CARTESIAN_POINT('Ctrl Pts',(-16.1742446642318,19.1756076137226,-18.2350898125817));
#39030=CARTESIAN_POINT('Ctrl Pts',(-16.1754068636011,19.0915515115639,-18.2392595269025));
#39031=CARTESIAN_POINT('Ctrl Pts',(-16.180714144804,19.0075207711868,-18.2434292412233));
#39032=CARTESIAN_POINT('Ctrl Pts',(-16.1901438433302,18.9239532195391,-18.2475989555441));
#39033=CARTESIAN_POINT('Ctrl Pts',(-16.1995732063072,18.8403886415836,-18.2517685214886));
#39034=CARTESIAN_POINT('Ctrl Pts',(-16.2131246425145,18.7572876766228,-18.2559380874331));
#39035=CARTESIAN_POINT('Ctrl Pts',(-16.2307236899663,18.675082361156,-18.2601076533775));
#39036=CARTESIAN_POINT('Ctrl Pts',(-16.2489414982118,18.5899868082275,-18.264423816116));
#39037=CARTESIAN_POINT('Ctrl Pts',(-16.2714967310844,18.5058515744436,-18.2687399788544));
#39038=CARTESIAN_POINT('Ctrl Pts',(-16.2982497538328,18.4231416762538,-18.2730561415928));
#39039=CARTESIAN_POINT('Ctrl Pts',(-16.3241312996847,18.3431260442804,-18.2772317057849));
#39040=CARTESIAN_POINT('Ctrl Pts',(-16.3539411382346,18.2644447370891,-18.281407269977));
#39041=CARTESIAN_POINT('Ctrl Pts',(-16.387503456575,18.1874991589185,-18.2855828341691));
#39042=CARTESIAN_POINT('Ctrl Pts',(-16.4227609278166,18.1066672425414,-18.2899692961806));
#39043=CARTESIAN_POINT('Ctrl Pts',(-16.4621596558343,18.0277515290339,-18.2943557581922));
#39044=CARTESIAN_POINT('Ctrl Pts',(-16.5054419382127,17.9511869324211,-18.2987422202037));
#39045=CARTESIAN_POINT('Ctrl Pts',(-16.548724220591,17.8746223358082,-18.3031286822153));
#39046=CARTESIAN_POINT('Ctrl Pts',(-16.5958896819152,17.8004093049792,-18.3075151442268));
#39047=CARTESIAN_POINT('Ctrl Pts',(-16.6466304638567,17.7289445288449,-18.3119016062384));
#39048=CARTESIAN_POINT('Ctrl Pts',(-16.6950365872103,17.6607679529895,-18.3160862406309));
#39049=CARTESIAN_POINT('Ctrl Pts',(-16.7468764264203,17.5948385205843,-18.3202708750235));
#39050=CARTESIAN_POINT('Ctrl Pts',(-16.8019140327136,17.5315227554341,-18.324455509416));
#39051=CARTESIAN_POINT('Ctrl Pts',(-16.8568732997865,17.4682971124385,-18.3286341874995));
#39052=CARTESIAN_POINT('Ctrl Pts',(-16.9150209937605,17.4076780913738,-18.3328128655829));
#39053=CARTESIAN_POINT('Ctrl Pts',(-16.9760786251332,17.3500022998976,-18.3369915436664));
#39054=CARTESIAN_POINT('Ctrl Pts',(-17.0382306706762,17.2912927113013,-18.3412451215519));
#39055=CARTESIAN_POINT('Ctrl Pts',(-17.1033977218496,17.2356332980397,-18.3454986994375));
#39056=CARTESIAN_POINT('Ctrl Pts',(-17.1712439260892,17.1833428659029,-18.3497522773231));
#39057=CARTESIAN_POINT('Ctrl Pts',(-17.2377747992588,17.132066185837,-18.3539233913005));
#39058=CARTESIAN_POINT('Ctrl Pts',(-17.3068814901404,17.0840293178158,-18.358094505278));
#39059=CARTESIAN_POINT('Ctrl Pts',(-17.3782123821184,17.0394936253377,-18.3622656192554));
#39060=CARTESIAN_POINT('Ctrl Pts',(-17.4495193383267,16.9949728772413,-18.3664353335753));
#39061=CARTESIAN_POINT('Ctrl Pts',(-17.5230486234685,16.9539512148435,-18.3706050478952));
#39062=CARTESIAN_POINT('Ctrl Pts',(-17.5984198264988,16.9166465683006,-18.3747747622151));
#39063=CARTESIAN_POINT('Ctrl Pts',(-17.6737883474984,16.879343249217,-18.3789443281587));
#39064=CARTESIAN_POINT('Ctrl Pts',(-17.7509982433954,16.8457568863071,-18.3831138941022));
#39065=CARTESIAN_POINT('Ctrl Pts',(-17.8296459350048,16.8160587219878,-18.3872834600458));
#39066=CARTESIAN_POINT('Ctrl Pts',(-17.9110587824491,16.78531640684,-18.3915996227853));
#39067=CARTESIAN_POINT('Ctrl Pts',(-17.9940119191525,16.7587409819327,-18.3959157855248));
#39068=CARTESIAN_POINT('Ctrl Pts',(-18.0780387582283,16.736466741122,-18.4002319482643));
#39069=CARTESIAN_POINT('Ctrl Pts',(-18.1593284318393,16.7149180813682,-18.4044075124555));
#39070=CARTESIAN_POINT('Ctrl Pts',(-18.241622459801,16.697394738803,-18.4085830766467));
#39071=CARTESIAN_POINT('Ctrl Pts',(-18.3244881604803,16.6839661550954,-18.412758640838));
#39072=CARTESIAN_POINT('Ctrl Pts',(-18.4115392107379,16.6698593255431,-18.4171451028516));
#39073=CARTESIAN_POINT('Ctrl Pts',(-18.4992206213763,16.6602718418454,-18.4215315648652));
#39074=CARTESIAN_POINT('Ctrl Pts',(-18.5870272090961,16.6552224277661,-18.4259180268789));
#39075=CARTESIAN_POINT('Ctrl Pts',(-18.6748337968158,16.6501730136867,-18.4303044888925));
#39076=CARTESIAN_POINT('Ctrl Pts',(-18.7627649809675,16.6496615965365,-18.4346909509062));
#39077=CARTESIAN_POINT('Ctrl Pts',(-18.8503205710793,16.6536440363642,-18.4390774129198));
#39078=CARTESIAN_POINT('Ctrl Pts',(-18.933847598669,16.6574432382305,-18.4432620473123));
#39079=CARTESIAN_POINT('Ctrl Pts',(-19.0173437395032,16.6653459878635,-18.4474466817047));
#39080=CARTESIAN_POINT('Ctrl Pts',(-19.1003730904697,16.6773522820685,-18.4516313160972));
#39081=CARTESIAN_POINT('Ctrl Pts',(-19.1832842594318,16.6893414867997,-18.4558099941806));
#39082=CARTESIAN_POINT('Ctrl Pts',(-19.2657295068654,16.7054225689875,-18.4599886722639));
#39083=CARTESIAN_POINT('Ctrl Pts',(-19.3472750579142,16.7255435623732,-18.4641673503473));
#39084=CARTESIAN_POINT('Ctrl Pts',(-19.4302822543744,16.7460252101083,-18.4684209282328));
#39085=CARTESIAN_POINT('Ctrl Pts',(-19.5123567014427,16.7706930025011,-18.4726745061184));
#39086=CARTESIAN_POINT('Ctrl Pts',(-19.5930485432788,16.7994371042225,-18.476928084004));
#39087=CARTESIAN_POINT('Ctrl Pts',(-19.6721760162895,16.8276239454375,-18.4810991979814));
#39088=CARTESIAN_POINT('Ctrl Pts',(-19.7499735613555,16.8597302905279,-18.4852703119587));
#39089=CARTESIAN_POINT('Ctrl Pts',(-19.8260310897313,16.8956019566692,-18.4894414259361));
#39090=CARTESIAN_POINT('Ctrl Pts',(-19.9020630962689,16.9314615857264,-18.4936111402558));
#39091=CARTESIAN_POINT('Ctrl Pts',(-19.9763558299785,16.9710838304486,-18.4977808545756));
#39092=CARTESIAN_POINT('Ctrl Pts',(-20.0485201368032,17.0142667868085,-18.5019505688954));
#39093=CARTESIAN_POINT('Ctrl Pts',(-20.120681875712,17.0574482065333,-18.5061201348388));
#39094=CARTESIAN_POINT('Ctrl Pts',(-20.1907149440075,17.1041898490219,-18.5102897007822));
#39095=CARTESIAN_POINT('Ctrl Pts',(-20.2582569041587,17.1542450583201,-18.5144592667256));
#39096=CARTESIAN_POINT('Ctrl Pts',(-20.3281735563287,17.2060601470437,-18.5187754294653));
#39097=CARTESIAN_POINT('Ctrl Pts',(-20.3954202425932,17.2614258339343,-18.5230915922049));
#39098=CARTESIAN_POINT('Ctrl Pts',(-20.4596314884394,17.3200224839765,-18.5274077549445));
#39099=CARTESIAN_POINT('Ctrl Pts',(-20.5217510596867,17.3767103542892,-18.5315833191356));
#39100=CARTESIAN_POINT('Ctrl Pts',(-20.5810296141597,17.4364215555164,-18.5357588833267));
#39101=CARTESIAN_POINT('Ctrl Pts',(-20.637174560043,17.4988298583361,-18.5399344475178));
#39102=CARTESIAN_POINT('Ctrl Pts',(-20.6961552536978,17.5643902561997,-18.5443209095317));
#39103=CARTESIAN_POINT('Ctrl Pts',(-20.7516770948088,17.6329269235823,-18.5487073715456));
#39104=CARTESIAN_POINT('Ctrl Pts',(-20.8034508935155,17.7040252160943,-18.5530938335595));
#39105=CARTESIAN_POINT('Ctrl Pts',(-20.8552246922223,17.7751235086063,-18.5574802955734));
#39106=CARTESIAN_POINT('Ctrl Pts',(-20.9032501953501,17.8487828986679,-18.5618667575873));
#39107=CARTESIAN_POINT('Ctrl Pts',(-20.9472937739972,17.9245589131308,-18.5662532196012));
#39108=CARTESIAN_POINT('Ctrl Pts',(-20.9909726387699,17.9997074453438,-18.5706033584188));
#39109=CARTESIAN_POINT('Ctrl Pts',(-21.0308877830075,18.0771985084606,-18.5749534972363));
#39110=CARTESIAN_POINT('Ctrl Pts',(-21.0667913726612,18.1566355413627,-18.5793036360538));
#39111=CARTESIAN_POINT('Ctrl Pts',(-21.1039225287098,18.2387885765656,-18.5838025088636));
#39112=CARTESIAN_POINT('Ctrl Pts',(-21.1367625751612,18.3230227236645,-18.5883013816734));
#39113=CARTESIAN_POINT('Ctrl Pts',(-21.1650869626505,18.4088677290927,-18.5928002544832));
#39114=CARTESIAN_POINT('Ctrl Pts',(-21.1923645588302,18.4915401396792,-18.5971328613513));
#39115=CARTESIAN_POINT('Ctrl Pts',(-21.2154541944225,18.5757060184776,-18.6014654682194));
#39116=CARTESIAN_POINT('Ctrl Pts',(-21.234202937817,18.6609224875245,-18.6057980750875));
#39117=CARTESIAN_POINT('Ctrl Pts',(-21.2529274817652,18.7460289656604,-18.6101250897574));
#39118=CARTESIAN_POINT('Ctrl Pts',(-21.2673221897251,18.8321829392873,-18.6144521044274));
#39119=CARTESIAN_POINT('Ctrl Pts',(-21.2772839154183,18.9189265065526,-18.6187791190974));
#39120=CARTESIAN_POINT('Ctrl Pts',(-21.2872318317724,19.0055498264465,-18.6231001354881));
#39121=CARTESIAN_POINT('Ctrl Pts',(-21.2927589555479,19.0927607071587,-18.6274211518788));
#39122=CARTESIAN_POINT('Ctrl Pts',(-21.2938134141941,19.1800923227686,-18.6317421682696));
#39123=CARTESIAN_POINT('Ctrl Pts',(-21.2939393290371,19.1905207513303,-18.6322581487702));
#39124=CARTESIAN_POINT('Ctrl Pts',(-21.2940015277988,19.2009508929668,-18.6327741292709));
#39125=CARTESIAN_POINT('Ctrl Pts',(-21.2939999715072,19.2113819467094,-18.6332901097715));
#39126=CARTESIAN_POINT('Ctrl Pts',(-21.2898372017813,19.2113866752102,-18.6332903748237));
#39127=CARTESIAN_POINT('Ctrl Pts',(-21.2903732285223,19.6159817978459,-18.6533365919766));
#39128=CARTESIAN_POINT('Ctrl Pts',(-21.0089154443045,20.8754716727687,-18.7157747446901));
#39129=CARTESIAN_POINT('Ctrl Pts',(-19.2309397186665,22.0893674765224,-18.810203250608));
#39130=CARTESIAN_POINT('Ctrl Pts',(-17.688669459474,21.6276028702836,-18.884585539373));
#39131=CARTESIAN_POINT('Ctrl Pts',(-17.1746506311398,21.2408837946621,-18.9165758925774));
#39132=CARTESIAN_POINT('',(-21.2939999971965,19.2111198080496,-18.5667098901964));
#39133=CARTESIAN_POINT('Ctrl Pts',(-21.2939999971965,19.2111198086917,-18.5667098902285));
#39134=CARTESIAN_POINT('Ctrl Pts',(-21.2939996986147,19.2174997239769,-18.5670291853155));
#39135=CARTESIAN_POINT('Ctrl Pts',(-21.2939755504833,19.223879573923,-18.5673484804024));
#39136=CARTESIAN_POINT('Ctrl Pts',(-21.2939275539577,19.2302592442234,-18.5676677754894));
#39137=CARTESIAN_POINT('Ctrl Pts',(-21.2932985185608,19.31387026376,-18.5718524098819));
#39138=CARTESIAN_POINT('Ctrl Pts',(-21.2885677156651,19.3976060296583,-18.5760370442745));
#39139=CARTESIAN_POINT('Ctrl Pts',(-21.2797186185528,19.4810309522135,-18.580221678667));
#39140=CARTESIAN_POINT('Ctrl Pts',(-21.2708821170351,19.5643371297175,-18.5844003567505));
#39141=CARTESIAN_POINT('Ctrl Pts',(-21.2579390129528,19.6473328891638,-18.5885790348339));
#39142=CARTESIAN_POINT('Ctrl Pts',(-21.2409247859828,19.7295827970778,-18.5927577129174));
#39143=CARTESIAN_POINT('Ctrl Pts',(-21.2236055912197,19.8133069754917,-18.5970112908029));
#39144=CARTESIAN_POINT('Ctrl Pts',(-21.2020678918843,19.8962578184688,-18.6012648686885));
#39145=CARTESIAN_POINT('Ctrl Pts',(-21.1764043852928,19.9779816286603,-18.605518446574));
#39146=CARTESIAN_POINT('Ctrl Pts',(-21.1512384158585,20.0581210633086,-18.6096895605515));
#39147=CARTESIAN_POINT('Ctrl Pts',(-21.1221053294156,20.1370801583403,-18.613860674529));
#39148=CARTESIAN_POINT('Ctrl Pts',(-21.0891436468889,20.2144432731942,-18.6180317885065));
#39149=CARTESIAN_POINT('Ctrl Pts',(-21.0561930249731,20.2917804281078,-18.6222015028263));
#39150=CARTESIAN_POINT('Ctrl Pts',(-21.0194165386216,20.3675222435798,-18.6263712171462));
#39151=CARTESIAN_POINT('Ctrl Pts',(-20.9790011895033,20.4412721890413,-18.6305409314661));
#39152=CARTESIAN_POINT('Ctrl Pts',(-20.9385872785366,20.5150195101634,-18.6347104974097));
#39153=CARTESIAN_POINT('Ctrl Pts',(-20.8945349840829,20.5867746991834,-18.6388800633533));
#39154=CARTESIAN_POINT('Ctrl Pts',(-20.8470770406692,20.6561662258013,-18.6430496292968));
#39155=CARTESIAN_POINT('Ctrl Pts',(-20.7979505344985,20.7279974729093,-18.6473657920363));
#39156=CARTESIAN_POINT('Ctrl Pts',(-20.7451747360215,20.7972953169815,-18.6516819547758));
#39157=CARTESIAN_POINT('Ctrl Pts',(-20.6890551911697,20.863682425477,-18.6559981175153));
#39158=CARTESIAN_POINT('Ctrl Pts',(-20.634763734602,20.9279069808801,-18.6601736817066));
#39159=CARTESIAN_POINT('Ctrl Pts',(-20.5773433873057,20.9894072108732,-18.6643492458978));
#39160=CARTESIAN_POINT('Ctrl Pts',(-20.517109048565,21.0478783631274,-18.668524810089));
#39161=CARTESIAN_POINT('Ctrl Pts',(-20.4538324165451,21.1093027543023,-18.6729112721026));
#39162=CARTESIAN_POINT('Ctrl Pts',(-20.3874504923528,21.1673836440657,-18.6772977341163));
#39163=CARTESIAN_POINT('Ctrl Pts',(-20.3183666557521,21.2218163268038,-18.6816841961299));
#39164=CARTESIAN_POINT('Ctrl Pts',(-20.2492828191514,21.276249009542,-18.6860706581436));
#39165=CARTESIAN_POINT('Ctrl Pts',(-20.1774975877418,21.327033212256,-18.6904571201572));
#39166=CARTESIAN_POINT('Ctrl Pts',(-20.1034462555222,21.3739186191894,-18.6948435821709));
#39167=CARTESIAN_POINT('Ctrl Pts',(-20.032802134896,21.4186467590315,-18.6990282165633));
#39168=CARTESIAN_POINT('Ctrl Pts',(-19.9598329133702,21.459993484366,-18.7032128509558));
#39169=CARTESIAN_POINT('Ctrl Pts',(-19.8848959073541,21.497709122393,-18.7073974853483));
#39170=CARTESIAN_POINT('Ctrl Pts',(-19.8100655648908,21.5353710768775,-18.7115761634316));
#39171=CARTESIAN_POINT('Ctrl Pts',(-19.733273408809,21.5694120050826,-18.715754841515));
#39172=CARTESIAN_POINT('Ctrl Pts',(-19.654904774228,21.5996260479204,-18.7199335195984));
#39173=CARTESIAN_POINT('Ctrl Pts',(-19.5751314381808,21.630381655767,-18.7241870974839));
#39174=CARTESIAN_POINT('Ctrl Pts',(-19.493724958338,21.6571715770569,-18.7284406753695));
#39175=CARTESIAN_POINT('Ctrl Pts',(-19.41111699767,21.6798281777933,-18.7326942532551));
#39176=CARTESIAN_POINT('Ctrl Pts',(-19.3301105535301,21.7020455361098,-18.7368653672325));
#39177=CARTESIAN_POINT('Ctrl Pts',(-19.2479492630204,21.7202882813848,-18.7410364812098));
#39178=CARTESIAN_POINT('Ctrl Pts',(-19.1650575928257,21.734447909442,-18.7452075951871));
#39179=CARTESIAN_POINT('Ctrl Pts',(-19.0821937377315,21.7486027860993,-18.7493773095069));
#39180=CARTESIAN_POINT('Ctrl Pts',(-18.9986004427839,21.7586771892408,-18.7535470238267));
#39181=CARTESIAN_POINT('Ctrl Pts',(-18.9147123478954,21.7646137232005,-18.7577167381465));
#39182=CARTESIAN_POINT('Ctrl Pts',(-18.8308272381054,21.7705500459129,-18.7618863040899));
#39183=CARTESIAN_POINT('Ctrl Pts',(-18.7466478081773,21.7723487605766,-18.7660558700333));
#39184=CARTESIAN_POINT('Ctrl Pts',(-18.6626124310825,21.7700044577929,-18.7702254359768));
#39185=CARTESIAN_POINT('Ctrl Pts',(-18.5756224737711,21.7675777322146,-18.7745415987164));
#39186=CARTESIAN_POINT('Ctrl Pts',(-18.4887874147817,21.7607112463061,-18.778857761456));
#39187=CARTESIAN_POINT('Ctrl Pts',(-18.4025899172848,21.749457672894,-18.7831739241957));
#39188=CARTESIAN_POINT('Ctrl Pts',(-18.3192002942283,21.7385706834556,-18.7873494883867));
#39189=CARTESIAN_POINT('Ctrl Pts',(-18.2364077885004,21.7235781663988,-18.7915250525778));
#39190=CARTESIAN_POINT('Ctrl Pts',(-18.1546390975914,21.7045799455322,-18.7957006167689));
#39191=CARTESIAN_POINT('Ctrl Pts',(-18.0687404644519,21.6846221696844,-18.8000870787828));
#39192=CARTESIAN_POINT('Ctrl Pts',(-17.9839723511224,21.6602435606427,-18.8044735407967));
#39193=CARTESIAN_POINT('Ctrl Pts',(-17.9008093086191,21.6316183655827,-18.8088600028106));
#39194=CARTESIAN_POINT('Ctrl Pts',(-17.8176462661158,21.6029931705227,-18.8132464648245));
#39195=CARTESIAN_POINT('Ctrl Pts',(-17.7360888041544,21.5701216768946,-18.8176329268384));
#39196=CARTESIAN_POINT('Ctrl Pts',(-17.6565830150584,21.5332344068933,-18.8220193888523));
#39197=CARTESIAN_POINT('Ctrl Pts',(-17.5807293782392,21.4980415786259,-18.8262043557623));
#39198=CARTESIAN_POINT('Ctrl Pts',(-17.5064606949712,21.4590628106661,-18.8303893226724));
#39199=CARTESIAN_POINT('Ctrl Pts',(-17.4341804046275,21.4164634477782,-18.8345742895824));
#39200=CARTESIAN_POINT('Ctrl Pts',(-17.3620114350738,21.3739296932975,-18.8387528111141));
#39201=CARTESIAN_POINT('Ctrl Pts',(-17.2918251656452,21.3277866569804,-18.8429313326457));
#39202=CARTESIAN_POINT('Ctrl Pts',(-17.2240032215556,21.2782468960159,-18.8471098541774));
#39203=CARTESIAN_POINT('Ctrl Pts',(-17.207345913612,21.2660797565316,-18.848136113758));
#39204=CARTESIAN_POINT('Ctrl Pts',(-17.1908311129492,21.2537079425745,-18.8491623733387));
#39205=CARTESIAN_POINT('Ctrl Pts',(-17.1744642439897,21.2411350264762,-18.8501886329194));
#39206=CARTESIAN_POINT('Ctrl Pts',(-17.1744642439897,21.2411350264762,-18.0500683119931));
#39207=CARTESIAN_POINT('Ctrl Pts',(-17.1273612179385,21.2049508060252,-18.05303372425));
#39208=CARTESIAN_POINT('Ctrl Pts',(-17.0815714415894,21.1671673406356,-18.0559991365068));
#39209=CARTESIAN_POINT('Ctrl Pts',(-17.0372042845896,21.1278944415811,-18.0589645487637));
#39210=CARTESIAN_POINT('Ctrl Pts',(-16.9745956774138,21.0724745842853,-18.0631491831568));
#39211=CARTESIAN_POINT('Ctrl Pts',(-16.9145885551714,21.0138810328614,-18.06733381755));
#39212=CARTESIAN_POINT('Ctrl Pts',(-16.8575221052048,20.9523875818855,-18.0715184519431));
#39213=CARTESIAN_POINT('Ctrl Pts',(-16.8005368822663,20.8909816592257,-18.0756971300271));
#39214=CARTESIAN_POINT('Ctrl Pts',(-16.7464843277716,20.8266843701414,-18.0798758081111));
#39215=CARTESIAN_POINT('Ctrl Pts',(-16.6956693348425,20.759808606471,-18.0840544861951));
#39216=CARTESIAN_POINT('Ctrl Pts',(-16.6439435196862,20.6917341428008,-18.0883080640805));
#39217=CARTESIAN_POINT('Ctrl Pts',(-16.5955728353226,20.6209881765787,-18.0925616419659));
#39218=CARTESIAN_POINT('Ctrl Pts',(-16.5508383402299,20.5479387298264,-18.0968152198513));
#39219=CARTESIAN_POINT('Ctrl Pts',(-16.506971110616,20.4763054891424,-18.1009863338293));
#39220=CARTESIAN_POINT('Ctrl Pts',(-16.4666005905002,20.4024576962093,-18.1051574478073));
#39221=CARTESIAN_POINT('Ctrl Pts',(-16.4299490395871,20.3267729033367,-18.1093285617853));
#39222=CARTESIAN_POINT('Ctrl Pts',(-16.393309787456,20.2511135072274,-18.1134982761058));
#39223=CARTESIAN_POINT('Ctrl Pts',(-16.3603872264447,20.1736187490988,-18.1176679904262));
#39224=CARTESIAN_POINT('Ctrl Pts',(-16.3313573525109,20.0946901654238,-18.1218377047466));
#39225=CARTESIAN_POINT('Ctrl Pts',(-16.3023285115847,20.0157643903665,-18.1260072706907));
#39226=CARTESIAN_POINT('Ctrl Pts',(-16.2771922403253,19.9354053232569,-18.1301768366348));
#39227=CARTESIAN_POINT('Ctrl Pts',(-16.2560756369329,19.854032542659,-18.1343464025789));
#39228=CARTESIAN_POINT('Ctrl Pts',(-16.2342165998161,19.7697987954821,-18.1386625653178));
#39229=CARTESIAN_POINT('Ctrl Pts',(-16.2166652853052,19.6844792346862,-18.1429787280566));
#39230=CARTESIAN_POINT('Ctrl Pts',(-16.203505316394,19.5985521335794,-18.1472948907955));
#39231=CARTESIAN_POINT('Ctrl Pts',(-16.1907740320855,19.5154240987507,-18.1514704549872));
#39232=CARTESIAN_POINT('Ctrl Pts',(-16.1821523920334,19.4317279704213,-18.1556460191789));
#39233=CARTESIAN_POINT('Ctrl Pts',(-16.177663165104,19.3479013752812,-18.1598215833707));
#39234=CARTESIAN_POINT('Ctrl Pts',(-16.1729471979947,19.2598408981034,-18.1642080453831));
#39235=CARTESIAN_POINT('Ctrl Pts',(-16.172792072363,19.1716370118691,-18.1685945073955));
#39236=CARTESIAN_POINT('Ctrl Pts',(-16.1771623761343,19.0837940049179,-18.1729809694079));
#39237=CARTESIAN_POINT('Ctrl Pts',(-16.1815326799056,18.9959509979667,-18.1773674314203));
#39238=CARTESIAN_POINT('Ctrl Pts',(-16.1904282787084,18.9084694398441,-18.1817538934327));
#39239=CARTESIAN_POINT('Ctrl Pts',(-16.2037517912763,18.8218419315364,-18.1861403554451));
#39240=CARTESIAN_POINT('Ctrl Pts',(-16.216462269281,18.7392002832971,-18.190324989838));
#39241=CARTESIAN_POINT('Ctrl Pts',(-16.2332494562526,18.657028211755,-18.194509624231));
#39242=CARTESIAN_POINT('Ctrl Pts',(-16.2540667299568,18.5757591195989,-18.198694258624));
#39243=CARTESIAN_POINT('Ctrl Pts',(-16.2748543728486,18.4946057039363,-18.2028729367079));
#39244=CARTESIAN_POINT('Ctrl Pts',(-16.2996605951405,18.4143531565235,-18.2070516147918));
#39245=CARTESIAN_POINT('Ctrl Pts',(-16.3283873371772,18.3354272066433,-18.2112302928757));
#39246=CARTESIAN_POINT('Ctrl Pts',(-16.3576289854198,18.2550865658331,-18.2154838707611));
#39247=CARTESIAN_POINT('Ctrl Pts',(-16.3909330131971,18.1761210253964,-18.2197374486466));
#39248=CARTESIAN_POINT('Ctrl Pts',(-16.4281421038534,18.0989661143749,-18.223991026532));
#39249=CARTESIAN_POINT('Ctrl Pts',(-16.4646298236791,18.0233070018604,-18.2281621405099));
#39250=CARTESIAN_POINT('Ctrl Pts',(-16.5048723340166,17.9493893735374,-18.2323332544878));
#39251=CARTESIAN_POINT('Ctrl Pts',(-16.5486724780851,17.8776044765483,-18.2365043684657));
#39252=CARTESIAN_POINT('Ctrl Pts',(-16.5924579245922,17.8058436676747,-18.240674082786));
#39253=CARTESIAN_POINT('Ctrl Pts',(-16.6397983945156,17.7362145612029,-18.2448437971064));
#39254=CARTESIAN_POINT('Ctrl Pts',(-16.6904515225,17.6690824859586,-18.2490135114267));
#39255=CARTESIAN_POINT('Ctrl Pts',(-16.7411028480287,17.6019527995617,-18.2531830773707));
#39256=CARTESIAN_POINT('Ctrl Pts',(-16.7950663194821,17.5373203344385,-18.2573526433147));
#39257=CARTESIAN_POINT('Ctrl Pts',(-16.8520579335329,17.4755190699805,-18.2615222092586));
#39258=CARTESIAN_POINT('Ctrl Pts',(-16.9110533024286,17.4115449493023,-18.2658383719976));
#39259=CARTESIAN_POINT('Ctrl Pts',(-16.9732933572886,17.3506052113062,-18.2701545347366));
#39260=CARTESIAN_POINT('Ctrl Pts',(-17.0384212094895,17.2930290499668,-18.2744706974756));
#39261=CARTESIAN_POINT('Ctrl Pts',(-17.1014275287535,17.2373284260287,-18.2786462616672));
#39262=CARTESIAN_POINT('Ctrl Pts',(-17.167135997239,17.1847758643076,-18.2828218258589));
#39263=CARTESIAN_POINT('Ctrl Pts',(-17.2351909645112,17.1356273888438,-18.2869973900505));
#39264=CARTESIAN_POINT('Ctrl Pts',(-17.3066832263981,17.0839965407216,-18.2913838520632));
#39265=CARTESIAN_POINT('Ctrl Pts',(-17.3807647695955,17.0361230139113,-18.2957703140758));
#39266=CARTESIAN_POINT('Ctrl Pts',(-17.4569923995306,16.9922499941761,-18.3001567760885));
#39267=CARTESIAN_POINT('Ctrl Pts',(-17.5332200294657,16.948376974441,-18.3045432381012));
#39268=CARTESIAN_POINT('Ctrl Pts',(-17.6115931945082,16.9085046570798,-18.3089297001138));
#39269=CARTESIAN_POINT('Ctrl Pts',(-17.6916449845519,16.8728177954295,-18.3133161621265));
#39270=CARTESIAN_POINT('Ctrl Pts',(-17.7680134730662,16.8387729391863,-18.3175007965194));
#39271=CARTESIAN_POINT('Ctrl Pts',(-17.8461937671331,16.8084101229908,-18.3216854309124));
#39272=CARTESIAN_POINT('Ctrl Pts',(-17.9257962079479,16.7819247375776,-18.3258700653053));
#39273=CARTESIAN_POINT('Ctrl Pts',(-18.0052853445408,16.7554770508323,-18.3300487433892));
#39274=CARTESIAN_POINT('Ctrl Pts',(-18.0861921743122,16.7328959763057,-18.334227421473));
#39275=CARTESIAN_POINT('Ctrl Pts',(-18.1681056484765,16.714329500532,-18.3384060995568));
#39276=CARTESIAN_POINT('Ctrl Pts',(-18.2514873627979,16.6954302340229,-18.3426596774423));
#39277=CARTESIAN_POINT('Ctrl Pts',(-18.3359117243126,16.6806911015683,-18.3469132553277));
#39278=CARTESIAN_POINT('Ctrl Pts',(-18.4209273694984,16.6702155683666,-18.3511668332132));
#39279=CARTESIAN_POINT('Ctrl Pts',(-18.5042948205052,16.6599431238176,-18.355337947191));
#39280=CARTESIAN_POINT('Ctrl Pts',(-18.5882303557915,16.6537704962434,-18.3595090611689));
#39281=CARTESIAN_POINT('Ctrl Pts',(-18.6722982812007,16.6517436826497,-18.3636801751467));
#39282=CARTESIAN_POINT('Ctrl Pts',(-18.7563379968057,16.649717549173,-18.367849889467));
#39283=CARTESIAN_POINT('Ctrl Pts',(-18.8405095547889,16.6518344778738,-18.3720196037873));
#39284=CARTESIAN_POINT('Ctrl Pts',(-18.9243745836524,16.6580884234077,-18.3761893181075));
#39285=CARTESIAN_POINT('Ctrl Pts',(-19.0082366282384,16.6643421463994,-18.3803588840515));
#39286=CARTESIAN_POINT('Ctrl Pts',(-19.0917917066962,16.6747325584671,-18.3845284499954));
#39287=CARTESIAN_POINT('Ctrl Pts',(-19.1746052695965,16.6892016344672,-18.3886980159393));
#39288=CARTESIAN_POINT('Ctrl Pts',(-19.2603304552117,16.7041794253309,-18.3930141786784));
#39289=CARTESIAN_POINT('Ctrl Pts',(-19.3452604921649,16.723527937402,-18.3973303414174));
#39290=CARTESIAN_POINT('Ctrl Pts',(-19.4289254033766,16.7471252702822,-18.4016465041565));
#39291=CARTESIAN_POINT('Ctrl Pts',(-19.5098649389009,16.7699539225245,-18.405822068348));
#39292=CARTESIAN_POINT('Ctrl Pts',(-19.5896200744158,16.796758641008,-18.4099976325396));
#39293=CARTESIAN_POINT('Ctrl Pts',(-19.667783027385,16.8273789609571,-18.4141731967312));
#39294=CARTESIAN_POINT('Ctrl Pts',(-19.7498938053008,16.8595458404767,-18.418559658744));
#39295=CARTESIAN_POINT('Ctrl Pts',(-19.8302467994661,16.8959236625789,-18.4229461207568));
#39296=CARTESIAN_POINT('Ctrl Pts',(-19.9083976363224,16.9362714026064,-18.4273325827696));
#39297=CARTESIAN_POINT('Ctrl Pts',(-19.9865484731787,16.9766191426339,-18.4317190447824));
#39298=CARTESIAN_POINT('Ctrl Pts',(-20.0624966899236,17.0209364424643,-18.4361055067951));
#39299=CARTESIAN_POINT('Ctrl Pts',(-20.1358342086536,17.0689307080656,-18.4404919688079));
#39300=CARTESIAN_POINT('Ctrl Pts',(-20.2057039471168,17.1146555545475,-18.4446710160258));
#39301=CARTESIAN_POINT('Ctrl Pts',(-20.2734659150699,17.1638887348098,-18.4488500632436));
#39302=CARTESIAN_POINT('Ctrl Pts',(-20.3387454860834,17.2164093339998,-18.4530291104615));
#39303=CARTESIAN_POINT('Ctrl Pts',(-20.4039320790894,17.2688551278475,-18.4572022054423));
#39304=CARTESIAN_POINT('Ctrl Pts',(-20.4666429412498,17.3245787540421,-18.461375300423));
#39305=CARTESIAN_POINT('Ctrl Pts',(-20.5265316718114,17.3833156165374,-18.4655483954038));
#39306=CARTESIAN_POINT('Ctrl Pts',(-20.5870226816091,17.4426431743496,-18.4697634576868));
#39307=CARTESIAN_POINT('Ctrl Pts',(-20.6446340707896,17.5050446643085,-18.4739785199699));
#39308=CARTESIAN_POINT('Ctrl Pts',(-20.6990425114803,17.5702050926228,-18.4781935822529));
#39309=CARTESIAN_POINT('Ctrl Pts',(-20.7528122887529,17.6346006473008,-18.4823591668069));
#39310=CARTESIAN_POINT('Ctrl Pts',(-20.8034536124378,17.701690347722,-18.4865247513609));
#39311=CARTESIAN_POINT('Ctrl Pts',(-20.8506921231952,17.7711338758054,-18.4906903359149));
#39312=CARTESIAN_POINT('Ctrl Pts',(-20.8979149500342,17.84055434756,-18.4948545374302));
#39313=CARTESIAN_POINT('Ctrl Pts',(-20.9417369482813,17.9123267137653,-18.4990187389455));
#39314=CARTESIAN_POINT('Ctrl Pts',(-20.9819260328715,17.9860801859964,-18.5031829404608));
#39315=CARTESIAN_POINT('Ctrl Pts',(-21.0221139173364,18.0598314558035,-18.5073470176248));
#39316=CARTESIAN_POINT('Ctrl Pts',(-21.0586688839109,18.1355633083682,-18.5115110947889));
#39317=CARTESIAN_POINT('Ctrl Pts',(-21.0914046022626,18.2128799965779,-18.5156751719529));
#39318=CARTESIAN_POINT('Ctrl Pts',(-21.1248385440613,18.2918457802491,-18.5199280651399));
#39319=CARTESIAN_POINT('Ctrl Pts',(-21.1542882228968,18.3724643312946,-18.5241809583268));
#39320=CARTESIAN_POINT('Ctrl Pts',(-21.1796074785073,18.4542939401135,-18.5284338515138));
#39321=CARTESIAN_POINT('Ctrl Pts',(-21.2044336791702,18.5345300386761,-18.5326039259141));
#39322=CARTESIAN_POINT('Ctrl Pts',(-21.2252888283686,18.6159299801768,-18.5367740003144));
#39323=CARTESIAN_POINT('Ctrl Pts',(-21.2420864983912,18.6980651926534,-18.5409440747148));
#39324=CARTESIAN_POINT('Ctrl Pts',(-21.2593845777047,18.7826472458753,-18.545238377295));
#39325=CARTESIAN_POINT('Ctrl Pts',(-21.2723795196075,18.8680085473307,-18.5495326798753));
#39326=CARTESIAN_POINT('Ctrl Pts',(-21.2810343673868,18.9536754357808,-18.5538269824556));
#39327=CARTESIAN_POINT('Ctrl Pts',(-21.2896892151661,19.0393423242309,-18.5581212850358));
#39328=CARTESIAN_POINT('Ctrl Pts',(-21.2940040128973,19.125314270194,-18.5624155876161));
#39329=CARTESIAN_POINT('Ctrl Pts',(-21.2939999971965,19.2111198080496,-18.5667098901964));
#39330=CARTESIAN_POINT('Origin',(-18.734,19.211,1.76670989022852));
#39331=CARTESIAN_POINT('',(-17.1762220931371,21.2388106152247,-17.2500265334082));
#39332=CARTESIAN_POINT('',(-17.1735447521835,21.2423105972199,-17.3168006939262));
#39333=CARTESIAN_POINT('',(-17.1744642439897,21.2411350264762,1.76670989022852));
#39334=CARTESIAN_POINT('',(-21.2939989159607,19.2086440968075,-17.8332901097715));
#39335=CARTESIAN_POINT('Ctrl Pts',(-17.1735447521834,21.2423105972199,-17.3168006939262));
#39336=CARTESIAN_POINT('Ctrl Pts',(-16.6213792194418,20.8094283882808,-17.3517574491069));
#39337=CARTESIAN_POINT('Ctrl Pts',(-15.7867860156331,19.3312717594939,-17.4291061398481));
#39338=CARTESIAN_POINT('Ctrl Pts',(-16.8703561089868,16.8256020863163,-17.5488467661498));
#39339=CARTESIAN_POINT('Ctrl Pts',(-19.7309870566021,16.3527997676692,-17.6760225728313));
#39340=CARTESIAN_POINT('Ctrl Pts',(-21.1817726888933,17.9552739588088,-17.7708370080137));
#39341=CARTESIAN_POINT('Ctrl Pts',(-21.2957665006941,19.0070072439541,-17.8232595076358));
#39342=CARTESIAN_POINT('Ctrl Pts',(-21.2939118038754,19.2086434116094,-17.8332900716974));
#39343=CARTESIAN_POINT('Ctrl Pts',(-21.2939989159607,19.2086440968075,-17.8332901097715));
#39344=CARTESIAN_POINT('Ctrl Pts',(-21.2940751741219,19.2915086264566,-17.837412174938));
#39345=CARTESIAN_POINT('Ctrl Pts',(-21.290123839502,19.3744847533444,-17.8415342401044));
#39346=CARTESIAN_POINT('Ctrl Pts',(-21.2821391268744,19.457144246514,-17.8456563052709));
#39347=CARTESIAN_POINT('Ctrl Pts',(-21.2741597741335,19.5397482529613,-17.8497756034244));
#39348=CARTESIAN_POINT('Ctrl Pts',(-21.262152459652,19.6220355783688,-17.8538949015779));
#39349=CARTESIAN_POINT('Ctrl Pts',(-21.2461634417033,19.7035797825424,-17.8580141997315));
#39350=CARTESIAN_POINT('Ctrl Pts',(-21.2301800733889,19.7850951735057,-17.862132042353));
#39351=CARTESIAN_POINT('Ctrl Pts',(-21.2102178848107,19.8658675009386,-17.8662498849744));
#39352=CARTESIAN_POINT('Ctrl Pts',(-21.1863745538874,19.9454787590158,-17.8703677275959));
#39353=CARTESIAN_POINT('Ctrl Pts',(-21.1625320679642,20.0250871956953,-17.8744854242823));
#39354=CARTESIAN_POINT('Ctrl Pts',(-21.1348088500427,20.1035341923717,-17.8786031209688));
#39355=CARTESIAN_POINT('Ctrl Pts',(-21.1033525053491,20.1804166830605,-17.8827208176552));
#39356=CARTESIAN_POINT('Ctrl Pts',(-21.0718661219911,20.2573725912857,-17.8868424464612));
#39357=CARTESIAN_POINT('Ctrl Pts',(-21.0366396717685,20.3327605713694,-17.8909640752672));
#39358=CARTESIAN_POINT('Ctrl Pts',(-20.9978687619912,20.4061979871471,-17.8950857040732));
#39359=CARTESIAN_POINT('Ctrl Pts',(-20.9590794967267,20.4796701707327,-17.8992092842006));
#39360=CARTESIAN_POINT('Ctrl Pts',(-20.9167426732501,20.551189545137,-17.9033328643279));
#39361=CARTESIAN_POINT('Ctrl Pts',(-20.8710983794445,20.6204007650685,-17.9074564444553));
#39362=CARTESIAN_POINT('Ctrl Pts',(-20.8253741239694,20.6897332322411,-17.9115872484506));
#39363=CARTESIAN_POINT('Ctrl Pts',(-20.7763311058832,20.7567490876314,-17.9157180524459));
#39364=CARTESIAN_POINT('Ctrl Pts',(-20.7242507920073,20.8211247730888,-17.9198488564413));
#39365=CARTESIAN_POINT('Ctrl Pts',(-20.6800170723896,20.8758014024867,-17.9233572996922));
#39366=CARTESIAN_POINT('Ctrl Pts',(-20.6335931281538,20.9285739549631,-17.9268657429431));
#39367=CARTESIAN_POINT('Ctrl Pts',(-20.5851713910723,20.9792659530951,-17.9303741861941));
#39368=CARTESIAN_POINT('Ctrl Pts',(-20.5274172101246,21.0397279482481,-17.9345588205871));
#39369=CARTESIAN_POINT('Ctrl Pts',(-20.4665902688467,21.0974699797564,-17.9387434549801));
#39370=CARTESIAN_POINT('Ctrl Pts',(-20.4029770272298,21.1521634868241,-17.9429280893731));
#39371=CARTESIAN_POINT('Ctrl Pts',(-20.3394543311886,21.2067791444542,-17.947106767457));
#39372=CARTESIAN_POINT('Ctrl Pts',(-20.2731535582846,21.2583545993042,-17.9512854455408));
#39373=CARTESIAN_POINT('Ctrl Pts',(-20.2043989371767,21.3065970427421,-17.9554641236247));
#39374=CARTESIAN_POINT('Ctrl Pts',(-20.1344119388974,21.3557041973082,-17.9597177015102));
#39375=CARTESIAN_POINT('Ctrl Pts',(-20.0618825897101,21.4013573280785,-17.9639712793956));
#39376=CARTESIAN_POINT('Ctrl Pts',(-19.9871893049689,21.4432895345164,-17.9682248572811));
#39377=CARTESIAN_POINT('Ctrl Pts',(-19.9139440953056,21.4844088033079,-17.972395971259));
#39378=CARTESIAN_POINT('Ctrl Pts',(-19.8386185251855,21.5219498994727,-17.9765670852369));
#39379=CARTESIAN_POINT('Ctrl Pts',(-19.7615983036838,21.555705040355,-17.9807381992148));
#39380=CARTESIAN_POINT('Ctrl Pts',(-19.6846039270612,21.5894488543738,-17.9849079135351));
#39381=CARTESIAN_POINT('Ctrl Pts',(-19.6059164494116,21.619409051666,-17.9890776278554));
#39382=CARTESIAN_POINT('Ctrl Pts',(-19.5259437923522,21.6454249895519,-17.9932473421757));
#39383=CARTESIAN_POINT('Ctrl Pts',(-19.4459739810633,21.6714400016791,-17.9974169081197));
#39384=CARTESIAN_POINT('Ctrl Pts',(-19.3647195190225,21.6935108919569,-18.0015864740637));
#39385=CARTESIAN_POINT('Ctrl Pts',(-19.2826045027058,21.7115265644681,-18.0057560400077));
#39386=CARTESIAN_POINT('Ctrl Pts',(-19.1976024237129,21.7301756458007,-18.0100722027467));
#39387=CARTESIAN_POINT('Ctrl Pts',(-19.1116786655147,21.7444789277004,-18.0143883654857));
#39388=CARTESIAN_POINT('Ctrl Pts',(-19.0253143284886,21.7543709839536,-18.0187045282247));
#39389=CARTESIAN_POINT('Ctrl Pts',(-18.9417633006594,21.7639408075146,-18.0228800924163));
#39390=CARTESIAN_POINT('Ctrl Pts',(-18.857800430025,21.7693824000208,-18.0270556566079));
#39391=CARTESIAN_POINT('Ctrl Pts',(-18.7738638919265,21.7706896042529,-18.0312312207996));
#39392=CARTESIAN_POINT('Ctrl Pts',(-18.6856879188254,21.7720628322632,-18.0356176828122));
#39393=CARTESIAN_POINT('Ctrl Pts',(-18.5975415917828,21.7688730610124,-18.0400041448249));
#39394=CARTESIAN_POINT('Ctrl Pts',(-18.5099274935593,21.7611748002553,-18.0443906068375));
#39395=CARTESIAN_POINT('Ctrl Pts',(-18.4223133953359,21.7534765394983,-18.0487770688502));
#39396=CARTESIAN_POINT('Ctrl Pts',(-18.3352320899719,21.7412699451077,-18.0531635308629));
#39397=CARTESIAN_POINT('Ctrl Pts',(-18.2491721313432,21.7246710082613,-18.0575499928755));
#39398=CARTESIAN_POINT('Ctrl Pts',(-18.167067998592,21.7088350569539,-18.0617348270903));
#39399=CARTESIAN_POINT('Ctrl Pts',(-18.0855877575544,21.6889427479729,-18.0659196613052));
#39400=CARTESIAN_POINT('Ctrl Pts',(-18.005162792895,21.6650571153784,-18.07010449552));
#39401=CARTESIAN_POINT('Ctrl Pts',(-17.9248712290094,21.6412111018485,-18.0742823883563));
#39402=CARTESIAN_POINT('Ctrl Pts',(-17.8456318987017,21.6133850633005,-18.0784602811926));
#39403=CARTESIAN_POINT('Ctrl Pts',(-17.7678662694045,21.5816930663006,-18.0826381740289));
#39404=CARTESIAN_POINT('Ctrl Pts',(-17.6901757082992,21.5500316620051,-18.0868120338899));
#39405=CARTESIAN_POINT('Ctrl Pts',(-17.6139564476223,21.5145118802857,-18.0909858937509));
#39406=CARTESIAN_POINT('Ctrl Pts',(-17.5396142320322,21.4752973826942,-18.0951597536119));
#39407=CARTESIAN_POINT('Ctrl Pts',(-17.4653211999168,21.4361088287101,-18.0993308521222));
#39408=CARTESIAN_POINT('Ctrl Pts',(-17.3929031526805,21.3932306267404,-18.1035019506325));
#39409=CARTESIAN_POINT('Ctrl Pts',(-17.3227440412582,21.346873736651,-18.1076730491428));
#39410=CARTESIAN_POINT('Ctrl Pts',(-17.2720953304333,21.3134081371975,-18.1106842155898));
#39411=CARTESIAN_POINT('Ctrl Pts',(-17.2226234583587,21.2781306035241,-18.1136953820369));
#39412=CARTESIAN_POINT('Ctrl Pts',(-17.1744642439897,21.2411350264762,-18.1167065484839));
#39413=CARTESIAN_POINT('',(-21.2939990418858,19.2132148462352,-17.7667099127482));
#39414=CARTESIAN_POINT('Ctrl Pts',(-21.2939990418858,19.2132148462352,-17.7667099127482));
#39415=CARTESIAN_POINT('Ctrl Pts',(-21.2939112972768,19.3146332252686,-17.7717442924635));
#39416=CARTESIAN_POINT('Ctrl Pts',(-21.2877929815477,19.415787678657,-17.7767786721789));
#39417=CARTESIAN_POINT('Ctrl Pts',(-21.2757605528227,19.5160463769891,-17.7818130518942));
#39418=CARTESIAN_POINT('Ctrl Pts',(-21.2635573150943,19.6177283198494,-17.7869188982603));
#39419=CARTESIAN_POINT('Ctrl Pts',(-21.245270932932,19.7184889031551,-17.7920247446265));
#39420=CARTESIAN_POINT('Ctrl Pts',(-21.2210717431444,19.8176911442014,-17.7971305909926));
#39421=CARTESIAN_POINT('Ctrl Pts',(-21.2092508709255,19.866149668042,-17.7996247057953));
#39422=CARTESIAN_POINT('Ctrl Pts',(-21.1960198419246,19.9142366801055,-17.8021188205981));
#39423=CARTESIAN_POINT('Ctrl Pts',(-21.1814026084241,19.9618797988219,-17.8046129354008));
#39424=CARTESIAN_POINT('Ctrl Pts',(-21.1568777637899,20.0418155872439,-17.8087975697939));
#39425=CARTESIAN_POINT('Ctrl Pts',(-21.1283869296254,20.1206973427815,-17.8129822041869));
#39426=CARTESIAN_POINT('Ctrl Pts',(-21.0960388974778,20.1981029565359,-17.8171668385799));
#39427=CARTESIAN_POINT('Ctrl Pts',(-21.0637369087501,20.27539839298,-17.8213455166639));
#39428=CARTESIAN_POINT('Ctrl Pts',(-21.0275888032569,20.3512214402681,-17.8255241947478));
#39429=CARTESIAN_POINT('Ctrl Pts',(-20.9877531601769,20.4251650188473,-17.8297028728318));
#39430=CARTESIAN_POINT('Ctrl Pts',(-20.947203491824,20.5004339829303,-17.8339564507172));
#39431=CARTESIAN_POINT('Ctrl Pts',(-20.9028329287837,20.5737549756818,-17.8382100286026));
#39432=CARTESIAN_POINT('Ctrl Pts',(-20.8548601014715,20.6447197878198,-17.8424636064881));
#39433=CARTESIAN_POINT('Ctrl Pts',(-20.8078173210281,20.714308808598,-17.846634720466));
#39434=CARTESIAN_POINT('Ctrl Pts',(-20.7573109732373,20.7816317931437,-17.850805834444));
#39435=CARTESIAN_POINT('Ctrl Pts',(-20.7035927080245,20.8463301087233,-17.8549769484219));
#39436=CARTESIAN_POINT('Ctrl Pts',(-20.6498924684943,20.9110067141582,-17.8591466627423));
#39437=CARTESIAN_POINT('Ctrl Pts',(-20.5929827456749,20.9730600461347,-17.8633163770627));
#39438=CARTESIAN_POINT('Ctrl Pts',(-20.5331561759619,21.0321636539581,-17.867486091383));
#39439=CARTESIAN_POINT('Ctrl Pts',(-20.4733317351351,21.0912651586215,-17.8716556573271));
#39440=CARTESIAN_POINT('Ctrl Pts',(-20.4105909816462,21.147416825124,-17.8758252232711));
#39441=CARTESIAN_POINT('Ctrl Pts',(-20.345263220069,21.2003292426476,-17.8799947892152));
#39442=CARTESIAN_POINT('Ctrl Pts',(-20.2776386149851,21.2551019954969,-17.8843109519541));
#39443=CARTESIAN_POINT('Ctrl Pts',(-20.2072421084911,21.3064031452814,-17.888627114693));
#39444=CARTESIAN_POINT('Ctrl Pts',(-20.134474432863,21.3539585537049,-17.8929432774319));
#39445=CARTESIAN_POINT('Ctrl Pts',(-20.0640771566147,21.3999648497009,-17.8971188416236));
#39446=CARTESIAN_POINT('Ctrl Pts',(-19.9914612509378,21.4424654946024,-17.9012944058153));
#39447=CARTESIAN_POINT('Ctrl Pts',(-19.9170156443951,21.4812585723032,-17.905469970007));
#39448=CARTESIAN_POINT('Ctrl Pts',(-19.8388099672434,21.5220109961371,-17.9098564320195));
#39449=CARTESIAN_POINT('Ctrl Pts',(-19.7585854263164,21.5586712286021,-17.9142428940321));
#39450=CARTESIAN_POINT('Ctrl Pts',(-19.6768157184723,21.5910627136699,-17.9186293560446));
#39451=CARTESIAN_POINT('Ctrl Pts',(-19.5950460106282,21.6234541987377,-17.9230158180572));
#39452=CARTESIAN_POINT('Ctrl Pts',(-19.5117317099373,21.6515768229132,-17.9274022800697));
#39453=CARTESIAN_POINT('Ctrl Pts',(-19.427361531773,21.6753152773656,-17.9317887420823));
#39454=CARTESIAN_POINT('Ctrl Pts',(-19.3468694922151,21.69796257593,-17.9359735770739));
#39455=CARTESIAN_POINT('Ctrl Pts',(-19.2651168916007,21.7167042021081,-17.9401584120656));
#39456=CARTESIAN_POINT('Ctrl Pts',(-19.1825176034779,21.7314031342963,-17.9443432470572));
#39457=CARTESIAN_POINT('Ctrl Pts',(-19.1000369486759,21.7460809551264,-17.9485220715749));
#39458=CARTESIAN_POINT('Ctrl Pts',(-19.0167124711172,21.756727535891,-17.9527008960926));
#39459=CARTESIAN_POINT('Ctrl Pts',(-18.9329723420235,21.7632558663092,-17.9568797206103));
#39460=CARTESIAN_POINT('Ctrl Pts',(-18.8493333890532,21.7697763090973,-17.9610534962073));
#39461=CARTESIAN_POINT('Ctrl Pts',(-18.7652802392241,21.7721883584653,-17.9652272718043));
#39462=CARTESIAN_POINT('Ctrl Pts',(-18.6812489272003,21.7704564509517,-17.9694010474014));
#39463=CARTESIAN_POINT('Ctrl Pts',(-18.5972730476195,21.7687256859154,-17.9735720697083));
#39464=CARTESIAN_POINT('Ctrl Pts',(-18.5133194358117,21.7628564016069,-17.9777430920153));
#39465=CARTESIAN_POINT('Ctrl Pts',(-18.4298258472869,21.7528650799799,-17.9819141143222));
#39466=CARTESIAN_POINT('Ctrl Pts',(-18.3463622898504,21.7428773520452,-17.9860836363902));
#39467=CARTESIAN_POINT('Ctrl Pts',(-18.2633588832453,21.7287705870398,-17.9902531584581));
#39468=CARTESIAN_POINT('Ctrl Pts',(-18.1812486084931,21.7106131499068,-17.9944226805261));
#39469=CARTESIAN_POINT('Ctrl Pts',(-18.0991432365396,21.6924567969531,-17.9985919536321));
#39470=CARTESIAN_POINT('Ctrl Pts',(-18.0179313390517,21.6702503538478,-18.0027612267382));
#39471=CARTESIAN_POINT('Ctrl Pts',(-17.9380347007106,21.6441130763545,-18.0069304998443));
#39472=CARTESIAN_POINT('Ctrl Pts',(-17.8580775669164,21.6179560084609,-18.0111029298049));
#39473=CARTESIAN_POINT('Ctrl Pts',(-17.7794381185932,21.5878623064786,-18.0152753597655));
#39474=CARTESIAN_POINT('Ctrl Pts',(-17.7025213244531,21.5540005851241,-18.0194477897261));
#39475=CARTESIAN_POINT('Ctrl Pts',(-17.6255715835556,21.520124359344,-18.0236220069172));
#39476=CARTESIAN_POINT('Ctrl Pts',(-17.5503463788393,21.482477103769,-18.0277962241083));
#39477=CARTESIAN_POINT('Ctrl Pts',(-17.477227106474,21.4412739504595,-18.0319704412993));
#39478=CARTESIAN_POINT('Ctrl Pts',(-17.4040091462788,21.4000151859594,-18.0361502923599));
#39479=CARTESIAN_POINT('Ctrl Pts',(-17.3329031825643,21.3551911865764,-18.0403301434204));
#39480=CARTESIAN_POINT('Ctrl Pts',(-17.2642621217254,21.3070607264974,-18.044509994481));
#39481=CARTESIAN_POINT('Ctrl Pts',(-17.2338360925851,21.2857262837746,-18.046362766985));
#39482=CARTESIAN_POINT('Ctrl Pts',(-17.2038939434596,21.2637427190746,-18.048215539489));
#39483=CARTESIAN_POINT('Ctrl Pts',(-17.1744642439897,21.2411350264762,-18.0500683119931));
#39484=CARTESIAN_POINT('Ctrl Pts',(-17.1762220931372,21.2388106152247,-17.2500265334081));
#39485=CARTESIAN_POINT('Ctrl Pts',(-16.9304195186111,21.0526898980001,-17.2653209251638));
#39486=CARTESIAN_POINT('Ctrl Pts',(-16.1279939956761,20.1920438763241,-17.3230072524799));
#39487=CARTESIAN_POINT('Ctrl Pts',(-15.9988187087053,17.9140516790705,-17.4230855153565));
#39488=CARTESIAN_POINT('Ctrl Pts',(-18.3440265352185,16.209131858296,-17.5502613220379));
#39489=CARTESIAN_POINT('Ctrl Pts',(-20.7784813956588,17.1540155580924,-17.6648027803286));
#39490=CARTESIAN_POINT('Ctrl Pts',(-21.2874613721703,18.6141143669069,-17.7369523030588));
#39491=CARTESIAN_POINT('Ctrl Pts',(-21.2923873719166,19.2132129984815,-17.7667098902285));
#39492=CARTESIAN_POINT('Origin',(-18.734,19.211,1.76670989022852));
#39493=CARTESIAN_POINT('',(-17.1744642439897,21.2411350264762,-16.4501666835217));
#39494=CARTESIAN_POINT('',(-17.1744642439897,21.2411350264762,-16.5166303489465));
#39495=CARTESIAN_POINT('',(-17.1744642439897,21.2411350264762,1.76670989022852));
#39496=CARTESIAN_POINT('',(-21.2942631180427,19.2118355653576,-17.0332901097715));
#39497=CARTESIAN_POINT('Ctrl Pts',(-17.1744642439897,21.2411350264762,-16.5166303489465));
#39498=CARTESIAN_POINT('Ctrl Pts',(-17.1078975357866,21.1899989393446,-16.5208151793057));
#39499=CARTESIAN_POINT('Ctrl Pts',(-17.0439434920722,21.1356584139567,-16.5250000096648));
#39500=CARTESIAN_POINT('Ctrl Pts',(-16.982907842272,21.0784250333396,-16.5291848400239));
#39501=CARTESIAN_POINT('Ctrl Pts',(-16.9719425040963,21.0681427904953,-16.5299366642487));
#39502=CARTESIAN_POINT('Ctrl Pts',(-16.961071256108,21.0577672665176,-16.5306884884735));
#39503=CARTESIAN_POINT('Ctrl Pts',(-16.9502957329767,21.047300380603,-16.5314403126983));
#39504=CARTESIAN_POINT('Ctrl Pts',(-16.8903194470162,20.9890419614915,-16.5356249470914));
#39505=CARTESIAN_POINT('Ctrl Pts',(-16.8330887583091,20.9277336646777,-16.5398095814844));
#39506=CARTESIAN_POINT('Ctrl Pts',(-16.7789298175349,20.8636646912292,-16.5439942158775));
#39507=CARTESIAN_POINT('Ctrl Pts',(-16.7248479653093,20.7996869120342,-16.5481728939614));
#39508=CARTESIAN_POINT('Ctrl Pts',(-16.6738294707906,20.7329566097132,-16.5523515720454));
#39509=CARTESIAN_POINT('Ctrl Pts',(-16.6261644175017,20.6638004533156,-16.5565302501293));
#39510=CARTESIAN_POINT('Ctrl Pts',(-16.577645002389,20.5934047225164,-16.5607838280147));
#39511=CARTESIAN_POINT('Ctrl Pts',(-16.5326007777018,20.520495651305,-16.5650374059002));
#39512=CARTESIAN_POINT('Ctrl Pts',(-16.4912954660574,20.4454538765921,-16.5692909837856));
#39513=CARTESIAN_POINT('Ctrl Pts',(-16.4507909384799,20.3718669331139,-16.5734620977636));
#39514=CARTESIAN_POINT('Ctrl Pts',(-16.4138818774498,20.2962296630071,-16.5776332117415));
#39515=CARTESIAN_POINT('Ctrl Pts',(-16.3807728287042,20.2189295016394,-16.5818043257195));
#39516=CARTESIAN_POINT('Ctrl Pts',(-16.3476748900196,20.1416552790873,-16.5859740400399));
#39517=CARTESIAN_POINT('Ctrl Pts',(-16.3183746121639,20.0627196959935,-16.5901437543602));
#39518=CARTESIAN_POINT('Ctrl Pts',(-16.2930292165598,19.9825320047744,-16.5943134686806));
#39519=CARTESIAN_POINT('Ctrl Pts',(-16.2676847228536,19.9023471669775,-16.5984830346247));
#39520=CARTESIAN_POINT('Ctrl Pts',(-16.2462949694201,19.820910748543,-16.6026526005687));
#39521=CARTESIAN_POINT('Ctrl Pts',(-16.2289674972205,19.7386477613126,-16.6068221665128));
#39522=CARTESIAN_POINT('Ctrl Pts',(-16.2110308124741,19.6534925089336,-16.6111383292517));
#39523=CARTESIAN_POINT('Ctrl Pts',(-16.1974474922546,19.5674519980823,-16.6154544919906));
#39524=CARTESIAN_POINT('Ctrl Pts',(-16.1882789321129,19.4810078600997,-16.6197706547295));
#39525=CARTESIAN_POINT('Ctrl Pts',(-16.1794090368535,19.3973796308195,-16.6239462189212));
#39526=CARTESIAN_POINT('Ctrl Pts',(-16.1746706763875,19.3133741398416,-16.6281217831129));
#39527=CARTESIAN_POINT('Ctrl Pts',(-16.1740663387713,19.2294295987024,-16.6322973473046));
#39528=CARTESIAN_POINT('Ctrl Pts',(-16.1734314774988,19.1412452183496,-16.6366838093171));
#39529=CARTESIAN_POINT('Ctrl Pts',(-16.1773592072922,19.0531286901045,-16.6410702713296));
#39530=CARTESIAN_POINT('Ctrl Pts',(-16.1857908120614,18.965582122686,-16.6454567333422));
#39531=CARTESIAN_POINT('Ctrl Pts',(-16.1942224168306,18.8780355552674,-16.6498431953547));
#39532=CARTESIAN_POINT('Ctrl Pts',(-16.2071577359856,18.7910595113906,-16.6542296573673));
#39533=CARTESIAN_POINT('Ctrl Pts',(-16.2244766916358,18.7051415565825,-16.6586161193798));
#39534=CARTESIAN_POINT('Ctrl Pts',(-16.2409987764637,18.6231768142361,-16.6628007537728));
#39535=CARTESIAN_POINT('Ctrl Pts',(-16.2615714655045,18.5418698437248,-16.6669853881659));
#39536=CARTESIAN_POINT('Ctrl Pts',(-16.2861281256042,18.4616514252084,-16.6711700225589));
#39537=CARTESIAN_POINT('Ctrl Pts',(-16.3106498323378,18.3815471876818,-16.6753487006429));
#39538=CARTESIAN_POINT('Ctrl Pts',(-16.3391441128498,18.3025288606374,-16.6795273787268));
#39539=CARTESIAN_POINT('Ctrl Pts',(-16.3714933068751,18.225017178172,-16.6837060568108));
#39540=CARTESIAN_POINT('Ctrl Pts',(-16.4044223369543,18.1461161545051,-16.6879596346962));
#39541=CARTESIAN_POINT('Ctrl Pts',(-16.4413457432405,18.0687767925294,-16.6922132125816));
#39542=CARTESIAN_POINT('Ctrl Pts',(-16.4820862183798,17.9934268727714,-16.6964667904671));
#39543=CARTESIAN_POINT('Ctrl Pts',(-16.5220368599101,17.9195377582413,-16.700637904445));
#39544=CARTESIAN_POINT('Ctrl Pts',(-16.5656576595125,17.8475620591661,-16.704809018423));
#39545=CARTESIAN_POINT('Ctrl Pts',(-16.6127335620837,17.7778814775568,-16.7089801324009));
#39546=CARTESIAN_POINT('Ctrl Pts',(-16.6597936678812,17.7082242779395,-16.7131498467213));
#39547=CARTESIAN_POINT('Ctrl Pts',(-16.7103063167567,17.6408610471355,-16.7173195610417));
#39548=CARTESIAN_POINT('Ctrl Pts',(-16.7640124931676,17.5761455040512,-16.721489275362));
#39549=CARTESIAN_POINT('Ctrl Pts',(-16.8177167584822,17.5114322638236,-16.7256588413061));
#39550=CARTESIAN_POINT('Ctrl Pts',(-16.8746140309481,17.4493668774532,-16.7298284072501));
#39551=CARTESIAN_POINT('Ctrl Pts',(-16.9344051527487,17.3902698207185,-16.7339979731942));
#39552=CARTESIAN_POINT('Ctrl Pts',(-16.9962984566316,17.3290949843729,-16.7383141359331));
#39553=CARTESIAN_POINT('Ctrl Pts',(-17.0612925164448,17.2711014650387,-16.742630298672));
#39554=CARTESIAN_POINT('Ctrl Pts',(-17.1290155886976,17.2166015845683,-16.7469464614109));
#39555=CARTESIAN_POINT('Ctrl Pts',(-17.194532588995,17.163877031972,-16.7511220256026));
#39556=CARTESIAN_POINT('Ctrl Pts',(-17.2626031281001,17.1144222417058,-16.7552975897943));
#39557=CARTESIAN_POINT('Ctrl Pts',(-17.3328600861969,17.0684765014246,-16.759473153986));
#39558=CARTESIAN_POINT('Ctrl Pts',(-17.4066655562273,17.0202101510273,-16.7638596159985));
#39559=CARTESIAN_POINT('Ctrl Pts',(-17.4828836173806,16.9758169447298,-16.7682460780111));
#39560=CARTESIAN_POINT('Ctrl Pts',(-17.5610602937787,16.9355192935185,-16.7726325400236));
#39561=CARTESIAN_POINT('Ctrl Pts',(-17.6392369701768,16.8952216423073,-16.7770190020362));
#39562=CARTESIAN_POINT('Ctrl Pts',(-17.7193717017408,16.8590197157385,-16.7814054640487));
#39563=CARTESIAN_POINT('Ctrl Pts',(-17.800989527137,16.8270764572814,-16.7857919260613));
#39564=CARTESIAN_POINT('Ctrl Pts',(-17.8788519953999,16.7966029554973,-16.7899765604543));
#39565=CARTESIAN_POINT('Ctrl Pts',(-17.9583538968788,16.7698914102528,-16.7941611948474));
#39566=CARTESIAN_POINT('Ctrl Pts',(-18.0390969463692,16.7471189667408,-16.7983458292404));
#39567=CARTESIAN_POINT('Ctrl Pts',(-18.1197250681227,16.7243789369834,-16.8025245073243));
#39568=CARTESIAN_POINT('Ctrl Pts',(-18.2015903898501,16.7055669958483,-16.8067031854083));
#39569=CARTESIAN_POINT('Ctrl Pts',(-18.2842754534886,16.6908119450594,-16.8108818634922));
#39570=CARTESIAN_POINT('Ctrl Pts',(-18.3684425874682,16.6757924205895,-16.8151354413777));
#39571=CARTESIAN_POINT('Ctrl Pts',(-18.4534586911852,16.66497683224,-16.8193890192631));
#39572=CARTESIAN_POINT('Ctrl Pts',(-18.5388680958069,16.6584476420716,-16.8236425971485));
#39573=CARTESIAN_POINT('Ctrl Pts',(-18.6226216724573,16.6520450329952,-16.8278137111265));
#39574=CARTESIAN_POINT('Ctrl Pts',(-18.7067529564691,16.6497641415373,-16.8319848251044));
#39575=CARTESIAN_POINT('Ctrl Pts',(-18.7908245916081,16.6516307484483,-16.8361559390824));
#39576=CARTESIAN_POINT('Ctrl Pts',(-18.874868015698,16.6534967290012,-16.8403256534027));
#39577=CARTESIAN_POINT('Ctrl Pts',(-18.95885137113,16.659507433716,-16.8444953677231));
#39578=CARTESIAN_POINT('Ctrl Pts',(-19.0423370360802,16.6696365328467,-16.8486650820435));
#39579=CARTESIAN_POINT('Ctrl Pts',(-19.1258197302521,16.6797652715406,-16.8528346479875));
#39580=CARTESIAN_POINT('Ctrl Pts',(-19.2088043125729,16.6940120570168,-16.8570042139316));
#39581=CARTESIAN_POINT('Ctrl Pts',(-19.2908593851772,16.7122988123547,-16.8611737798756));
#39582=CARTESIAN_POINT('Ctrl Pts',(-19.3757994129083,16.7312285074512,-16.8654899426145));
#39583=CARTESIAN_POINT('Ctrl Pts',(-19.4597428368619,16.7544874341396,-16.8698061053534));
#39584=CARTESIAN_POINT('Ctrl Pts',(-19.542225826085,16.781932068869,-16.8741222680924));
#39585=CARTESIAN_POINT('Ctrl Pts',(-19.62202194061,16.8084826975088,-16.878297832284));
#39586=CARTESIAN_POINT('Ctrl Pts',(-19.7004508845913,16.838950308513,-16.8824733964757));
#39587=CARTESIAN_POINT('Ctrl Pts',(-19.777112739986,16.8731557340834,-16.8866489606674));
#39588=CARTESIAN_POINT('Ctrl Pts',(-19.8576466034503,16.9090887943838,-16.8910354226799));
#39589=CARTESIAN_POINT('Ctrl Pts',(-19.9362296554815,16.9491469214587,-16.8954218846925));
#39590=CARTESIAN_POINT('Ctrl Pts',(-20.0124291551047,16.9930687802869,-16.899808346705));
#39591=CARTESIAN_POINT('Ctrl Pts',(-20.088628654728,17.036990639115,-16.9041948087175));
#39592=CARTESIAN_POINT('Ctrl Pts',(-20.1624441562133,17.0847758505361,-16.9085812707301));
#39593=CARTESIAN_POINT('Ctrl Pts',(-20.2334815623277,17.1361132454422,-16.9129677327426));
#39594=CARTESIAN_POINT('Ctrl Pts',(-20.3007008312569,17.1846913445463,-16.9171184300414));
#39595=CARTESIAN_POINT('Ctrl Pts',(-20.3656920487853,17.2366370916662,-16.9212691273401));
#39596=CARTESIAN_POINT('Ctrl Pts',(-20.4280939407347,17.2917173944502,-16.9254198246388));
#39597=CARTESIAN_POINT('Ctrl Pts',(-20.4904067758308,17.3467190893862,-16.9295645982704));
#39598=CARTESIAN_POINT('Ctrl Pts',(-20.5501372744549,17.4048461509353,-16.9337093719019));
#39599=CARTESIAN_POINT('Ctrl Pts',(-20.6069541187605,17.4658229691467,-16.9378541455335));
#39600=CARTESIAN_POINT('Ctrl Pts',(-20.6637057912848,17.5267298438773,-16.9419941649009));
#39601=CARTESIAN_POINT('Ctrl Pts',(-20.7175501324578,17.5904796396565,-16.9461341842684));
#39602=CARTESIAN_POINT('Ctrl Pts',(-20.7681909845745,17.6567583719782,-16.9502742036359));
#39603=CARTESIAN_POINT('Ctrl Pts',(-20.8188004163149,17.7229959813208,-16.9544116543072));
#39604=CARTESIAN_POINT('Ctrl Pts',(-20.8662100198437,17.7917590422704,-16.9585491049784));
#39605=CARTESIAN_POINT('Ctrl Pts',(-20.9101632231195,17.8626997269368,-16.9626865556497));
#39606=CARTESIAN_POINT('Ctrl Pts',(-20.9541028768145,17.9336185425138,-16.9668227308571));
#39607=CARTESIAN_POINT('Ctrl Pts',(-20.994587999437,18.0067132510727,-16.9709589060645));
#39608=CARTESIAN_POINT('Ctrl Pts',(-21.031405596239,18.0816074524906,-16.9750950812719));
#39609=CARTESIAN_POINT('Ctrl Pts',(-21.0682233367814,18.1565019463047,-16.9792312726275));
#39610=CARTESIAN_POINT('Ctrl Pts',(-21.1013733182381,18.2331955257884,-16.983367463983));
#39611=CARTESIAN_POINT('Ctrl Pts',(-21.1306893947115,18.3112889656799,-16.9875036553386));
#39612=CARTESIAN_POINT('Ctrl Pts',(-21.1600333335746,18.3894566266172,-16.9916437777855));
#39613=CARTESIAN_POINT('Ctrl Pts',(-21.1855359272154,18.4690263650883,-16.9957839002324));
#39614=CARTESIAN_POINT('Ctrl Pts',(-21.2070801670876,18.549581458411,-16.9999240226793));
#39615=CARTESIAN_POINT('Ctrl Pts',(-21.2286351815299,18.6301768384412,-17.0040662156583));
#39616=CARTESIAN_POINT('Ctrl Pts',(-21.2462278030767,18.7117580962757,-17.0082084086373));
#39617=CARTESIAN_POINT('Ctrl Pts',(-21.2597921942375,18.7938983438909,-17.0123506016163));
#39618=CARTESIAN_POINT('Ctrl Pts',(-21.2733789861849,18.8761742412481,-17.016499635181));
#39619=CARTESIAN_POINT('Ctrl Pts',(-21.2829242114339,18.95901050629,-17.0206486687457));
#39620=CARTESIAN_POINT('Ctrl Pts',(-21.2884139728529,19.0419755778182,-17.0247977023105));
#39621=CARTESIAN_POINT('Ctrl Pts',(-21.2921595270972,19.0985809841503,-17.0276285047975));
#39622=CARTESIAN_POINT('Ctrl Pts',(-21.2940183320645,19.1552463005707,-17.0304593072845));
#39623=CARTESIAN_POINT('Ctrl Pts',(-21.2939998636668,19.2118354794421,-17.0332901097715));
#39624=CARTESIAN_POINT('Ctrl Pts',(-21.2979002849781,19.2118367523804,-17.0332901097715));
#39625=CARTESIAN_POINT('Ctrl Pts',(-21.2980949927007,19.2575742464713,-17.0355745863224));
#39626=CARTESIAN_POINT('Ctrl Pts',(-21.2762381497003,20.1518505805258,-17.0802509984337));
#39627=CARTESIAN_POINT('Ctrl Pts',(-20.2331956316243,21.8407726550478,-17.1673193461055));
#39628=CARTESIAN_POINT('Ctrl Pts',(-18.1310916553567,21.8801180010893,-17.2595383976062));
#39629=CARTESIAN_POINT('Ctrl Pts',(-17.2909884426572,21.3343831391365,-17.3093655135464));
#39630=CARTESIAN_POINT('Ctrl Pts',(-17.1735447521834,21.2423105972199,-17.3168006939262));
#39631=CARTESIAN_POINT('',(-21.2938494856171,19.209803254918,-16.9667098397541));
#39632=CARTESIAN_POINT('Ctrl Pts',(-21.2903253208441,19.2098059207881,-16.9667098902285));
#39633=CARTESIAN_POINT('Ctrl Pts',(-21.2882103114883,19.7131225250721,-16.9916592919231));
#39634=CARTESIAN_POINT('Ctrl Pts',(-20.9008595718265,21.0746360886269,-17.0590006291781));
#39635=CARTESIAN_POINT('Ctrl Pts',(-18.9946006269605,22.075603620026,-17.153439510238));
#39636=CARTESIAN_POINT('Ctrl Pts',(-17.6117180668893,21.5685664086269,-17.2229289896033));
#39637=CARTESIAN_POINT('Ctrl Pts',(-17.1762220931372,21.2388106152247,-17.2500265334081));
#39638=CARTESIAN_POINT('Ctrl Pts',(-17.1744642439897,21.2411350264762,-16.4501666835217));
#39639=CARTESIAN_POINT('Ctrl Pts',(-17.1078207226257,21.189939932003,-16.4543368993101));
#39640=CARTESIAN_POINT('Ctrl Pts',(-17.0436640483384,21.1354316379633,-16.4585071150985));
#39641=CARTESIAN_POINT('Ctrl Pts',(-16.9823341196667,21.0778868856136,-16.4626773308869));
#39642=CARTESIAN_POINT('Ctrl Pts',(-16.9210150140795,21.0203522883665,-16.4668468107442));
#39643=CARTESIAN_POINT('Ctrl Pts',(-16.8625219983004,20.9597826122461,-16.4710162906016));
#39644=CARTESIAN_POINT('Ctrl Pts',(-16.8071598200507,20.8964930794675,-16.4751857704589));
#39645=CARTESIAN_POINT('Ctrl Pts',(-16.7517908046024,20.8331957304664,-16.4793557652448));
#39646=CARTESIAN_POINT('Ctrl Pts',(-16.6995536963249,20.7671782049408,-16.4835257600306));
#39647=CARTESIAN_POINT('Ctrl Pts',(-16.6507135780857,20.6987895295596,-16.4876957548164));
#39648=CARTESIAN_POINT('Ctrl Pts',(-16.6018209673368,20.6303273512197,-16.4918702314401));
#39649=CARTESIAN_POINT('Ctrl Pts',(-16.5563329029902,20.5594893105763,-16.4960447080638));
#39650=CARTESIAN_POINT('Ctrl Pts',(-16.5144713431402,20.4866537701814,-16.5002191846875));
#39651=CARTESIAN_POINT('Ctrl Pts',(-16.4725853567887,20.4137757297593,-16.5043960971463));
#39652=CARTESIAN_POINT('Ctrl Pts',(-16.4343302969003,20.3388982788379,-16.5085730096052));
#39653=CARTESIAN_POINT('Ctrl Pts',(-16.3998812075074,20.262422589891,-16.512749922064));
#39654=CARTESIAN_POINT('Ctrl Pts',(-16.3653738793192,20.1858176129984,-16.5169338959098));
#39655=CARTESIAN_POINT('Ctrl Pts',(-16.3346855367979,20.1076094313179,-16.5211178697556));
#39656=CARTESIAN_POINT('Ctrl Pts',(-16.3079422109483,20.0282169872081,-16.5253018436014));
#39657=CARTESIAN_POINT('Ctrl Pts',(-16.2918496144703,19.980443177262,-16.5278195185964));
#39658=CARTESIAN_POINT('Ctrl Pts',(-16.2771845117736,19.9322408260174,-16.5303371935914));
#39659=CARTESIAN_POINT('Ctrl Pts',(-16.2639654295305,19.8837029215676,-16.5328548685864));
#39660=CARTESIAN_POINT('Ctrl Pts',(-16.2419939573158,19.803027939797,-16.5370395029795));
#39661=CARTESIAN_POINT('Ctrl Pts',(-16.223938199736,19.7211252621465,-16.5412241373725));
#39662=CARTESIAN_POINT('Ctrl Pts',(-16.2099316900943,19.638409834854,-16.5454087717656));
#39663=CARTESIAN_POINT('Ctrl Pts',(-16.1959451169855,19.5558121427341,-16.5495874498495));
#39664=CARTESIAN_POINT('Ctrl Pts',(-16.1859964196337,19.4724044485338,-16.5537661279335));
#39665=CARTESIAN_POINT('Ctrl Pts',(-16.18016901464,19.3886155911377,-16.5579448060174));
#39666=CARTESIAN_POINT('Ctrl Pts',(-16.1742371575999,19.3033248786908,-16.5621983839028));
#39667=CARTESIAN_POINT('Ctrl Pts',(-16.1725759211884,19.2176396691377,-16.5664519617883));
#39668=CARTESIAN_POINT('Ctrl Pts',(-16.1752185615464,19.1320218370346,-16.5707055396737));
#39669=CARTESIAN_POINT('Ctrl Pts',(-16.1778099691644,19.0480638736762,-16.5748766536517));
#39670=CARTESIAN_POINT('Ctrl Pts',(-16.1845398497979,18.9641711795844,-16.5790477676296));
#39671=CARTESIAN_POINT('Ctrl Pts',(-16.1953870618677,18.8807813597822,-16.5832188816076));
#39672=CARTESIAN_POINT('Ctrl Pts',(-16.2062306340507,18.7974195222395,-16.5873885959279));
#39673=CARTESIAN_POINT('Ctrl Pts',(-16.221188734479,18.7145606796676,-16.5915583102483));
#39674=CARTESIAN_POINT('Ctrl Pts',(-16.2401883815475,18.6326371280316,-16.5957280245687));
#39675=CARTESIAN_POINT('Ctrl Pts',(-16.2591873525271,18.5507164915873,-16.5998975905127));
#39676=CARTESIAN_POINT('Ctrl Pts',(-16.2822274794424,18.4697315278527,-16.6040671564568));
#39677=CARTESIAN_POINT('Ctrl Pts',(-16.3091849959464,18.3901028102639,-16.6082367224008));
#39678=CARTESIAN_POINT('Ctrl Pts',(-16.337090305475,18.3076744451974,-16.6125528851397));
#39679=CARTESIAN_POINT('Ctrl Pts',(-16.3691934316988,18.2266999715504,-16.6168690478787));
#39680=CARTESIAN_POINT('Ctrl Pts',(-16.4053020683426,18.1476252104293,-16.6211852106176));
#39681=CARTESIAN_POINT('Ctrl Pts',(-16.4402344699457,18.0711263013346,-16.6253607748093));
#39682=CARTESIAN_POINT('Ctrl Pts',(-16.4789151719813,17.9964056357569,-16.629536339001));
#39683=CARTESIAN_POINT('Ctrl Pts',(-16.5211232637327,17.9238416763712,-16.6337119031926));
#39684=CARTESIAN_POINT('Ctrl Pts',(-16.5654631858581,17.8476126839014,-16.6380983652052));
#39685=CARTESIAN_POINT('Ctrl Pts',(-16.613695880029,17.7737644826753,-16.6424848272177));
#39686=CARTESIAN_POINT('Ctrl Pts',(-16.6655152292137,17.7026993824091,-16.6468712892303));
#39687=CARTESIAN_POINT('Ctrl Pts',(-16.7173345783984,17.6316342821429,-16.6512577512428));
#39688=CARTESIAN_POINT('Ctrl Pts',(-16.7727401579415,17.5633526854597,-16.6556442132553));
#39689=CARTESIAN_POINT('Ctrl Pts',(-16.8313804354227,17.4982131503051,-16.6600306752679));
#39690=CARTESIAN_POINT('Ctrl Pts',(-16.8873225868114,17.4360707817228,-16.6642153096609));
#39691=CARTESIAN_POINT('Ctrl Pts',(-16.9464165382124,17.3765563809787,-16.668399944054));
#39692=CARTESIAN_POINT('Ctrl Pts',(-17.0083856645508,17.3200068309768,-16.6725845784471));
#39693=CARTESIAN_POINT('Ctrl Pts',(-17.070266585508,17.2635377722601,-16.676763256531));
#39694=CARTESIAN_POINT('Ctrl Pts',(-17.1350142155921,17.2100254892842,-16.6809419346149));
#39695=CARTESIAN_POINT('Ctrl Pts',(-17.2023131209905,17.1597722445643,-16.6851206126989));
#39696=CARTESIAN_POINT('Ctrl Pts',(-17.2708183109012,17.108618246549,-16.6893741905843));
#39697=CARTESIAN_POINT('Ctrl Pts',(-17.3419668163953,17.0608416308408,-16.6936277684698));
#39698=CARTESIAN_POINT('Ctrl Pts',(-17.4153882749825,17.0167203645282,-16.6978813463552));
#39699=CARTESIAN_POINT('Ctrl Pts',(-17.4873863153249,16.9734544750586,-16.7020524603332));
#39700=CARTESIAN_POINT('Ctrl Pts',(-17.5615695514942,16.9337037154835,-16.7062235743111));
#39701=CARTESIAN_POINT('Ctrl Pts',(-17.6375585833825,16.8976871763798,-16.7103946882891));
#39702=CARTESIAN_POINT('Ctrl Pts',(-17.7135221164171,16.8616827229737,-16.7145644026094));
#39703=CARTESIAN_POINT('Ctrl Pts',(-17.7912898263828,16.8294101983213,-16.7187341169298));
#39704=CARTESIAN_POINT('Ctrl Pts',(-17.8704587172267,16.8010422300492,-16.7229038312502));
#39705=CARTESIAN_POINT('Ctrl Pts',(-17.9496247909019,16.7726752712311,-16.7270733971942));
#39706=CARTESIAN_POINT('Ctrl Pts',(-18.0301915129629,16.7482127469196,-16.7312429631382));
#39707=CARTESIAN_POINT('Ctrl Pts',(-18.1117382553311,16.7277782376273,-16.7354125290823));
#39708=CARTESIAN_POINT('Ctrl Pts',(-18.1961520805622,16.7066252761969,-16.7397286918212));
#39709=CARTESIAN_POINT('Ctrl Pts',(-18.2816156117521,16.6897889781385,-16.7440448545601));
#39710=CARTESIAN_POINT('Ctrl Pts',(-18.3676498921635,16.6773489588169,-16.748361017299));
#39711=CARTESIAN_POINT('Ctrl Pts',(-18.4508816149397,16.6653141718163,-16.7525365814907));
#39712=CARTESIAN_POINT('Ctrl Pts',(-18.5346470002632,16.6573936417868,-16.7567121456824));
#39713=CARTESIAN_POINT('Ctrl Pts',(-18.6185082461362,16.6536064724432,-16.7608877098741));
#39714=CARTESIAN_POINT('Ctrl Pts',(-18.7066051241772,16.6496280221792,-16.7652741718866));
#39715=CARTESIAN_POINT('Ctrl Pts',(-18.7948072172264,16.6502114543057,-16.7696606338992));
#39716=CARTESIAN_POINT('Ctrl Pts',(-18.8826105511364,16.6553171354624,-16.7740470959117));
#39717=CARTESIAN_POINT('Ctrl Pts',(-18.9704138850463,16.6604228166191,-16.7784335579242));
#39718=CARTESIAN_POINT('Ctrl Pts',(-19.0578178914166,16.6700506076701,-16.7828200199368));
#39719=CARTESIAN_POINT('Ctrl Pts',(-19.1443308019264,16.6840990060965,-16.7872064819493));
#39720=CARTESIAN_POINT('Ctrl Pts',(-19.2268631251808,16.6975010168866,-16.7913911163424));
#39721=CARTESIAN_POINT('Ctrl Pts',(-19.3088917529363,16.7149756618514,-16.7955757507354));
#39722=CARTESIAN_POINT('Ctrl Pts',(-19.389983688077,16.7364726914061,-16.7997603851285));
#39723=CARTESIAN_POINT('Ctrl Pts',(-19.4709601988852,16.7579391226001,-16.8039390632124));
#39724=CARTESIAN_POINT('Ctrl Pts',(-19.5510022244943,16.7834164491322,-16.8081177412964));
#39725=CARTESIAN_POINT('Ctrl Pts',(-19.6296848716229,16.8128030500508,-16.8122964193803));
#39726=CARTESIAN_POINT('Ctrl Pts',(-19.709777848653,16.842716384671,-16.8165499972657));
#39727=CARTESIAN_POINT('Ctrl Pts',(-19.7884617582361,16.8766804423688,-16.8208035751512));
#39728=CARTESIAN_POINT('Ctrl Pts',(-19.8653024038484,16.9145342652139,-16.8250571530366));
#39729=CARTESIAN_POINT('Ctrl Pts',(-19.9406533436033,16.9516542178375,-16.8292282670146));
#39730=CARTESIAN_POINT('Ctrl Pts',(-20.0142314204538,16.9925142474789,-16.8333993809925));
#39731=CARTESIAN_POINT('Ctrl Pts',(-20.0856470518142,17.0369139282627,-16.8375704949705));
#39732=CARTESIAN_POINT('Ctrl Pts',(-20.15703871897,17.081298710305,-16.8417402092909));
#39733=CARTESIAN_POINT('Ctrl Pts',(-20.2262689913884,17.129220541882,-16.8459099236112));
#39734=CARTESIAN_POINT('Ctrl Pts',(-20.2929745824343,17.1804340071488,-16.8500796379316));
#39735=CARTESIAN_POINT('Ctrl Pts',(-20.3596777998089,17.2316456500206,-16.8542492038757));
#39736=CARTESIAN_POINT('Ctrl Pts',(-20.4238561500595,17.2861484128726,-16.8584187698197));
#39737=CARTESIAN_POINT('Ctrl Pts',(-20.4851780435309,17.3436555058438,-16.8625883357638));
#39738=CARTESIAN_POINT('Ctrl Pts',(-20.5486559391278,17.4031844772611,-16.8669044985027));
#39739=CARTESIAN_POINT('Ctrl Pts',(-20.6090723898819,17.4659326132814,-16.8712206612416));
#39740=CARTESIAN_POINT('Ctrl Pts',(-20.6661012016731,17.5315402813722,-16.8755368239805));
#39741=CARTESIAN_POINT('Ctrl Pts',(-20.7212723059185,17.5950107865757,-16.8797123881722));
#39742=CARTESIAN_POINT('Ctrl Pts',(-20.7732728325617,17.6611569867929,-16.8838879523639));
#39743=CARTESIAN_POINT('Ctrl Pts',(-20.8218497444838,17.7296211003059,-16.8880635165556));
#39744=CARTESIAN_POINT('Ctrl Pts',(-20.8728801607464,17.8015431734344,-16.8924499785681));
#39745=CARTESIAN_POINT('Ctrl Pts',(-20.9201317067406,17.8760229761494,-16.8968364405807));
#39746=CARTESIAN_POINT('Ctrl Pts',(-20.9633649162028,17.952615293162,-16.9012229025932));
#39747=CARTESIAN_POINT('Ctrl Pts',(-21.0065981256651,18.0292076101745,-16.9056093646057));
#39748=CARTESIAN_POINT('Ctrl Pts',(-21.0458128079223,18.1079118882385,-16.9099958266183));
#39749=CARTESIAN_POINT('Ctrl Pts',(-21.0808281256647,18.1882596866315,-16.9143822886308));
#39750=CARTESIAN_POINT('Ctrl Pts',(-21.117652895614,18.2727595393394,-16.9189954255354));
#39751=CARTESIAN_POINT('Ctrl Pts',(-21.1499518315869,18.3593459986734,-16.92360856244));
#39752=CARTESIAN_POINT('Ctrl Pts',(-21.1775079602936,18.4475415217695,-16.9282216993445));
#39753=CARTESIAN_POINT('Ctrl Pts',(-21.204985218715,18.5354846144123,-16.9328216326737));
#39754=CARTESIAN_POINT('Ctrl Pts',(-21.2277466226995,18.6250273148932,-16.9374215660029));
#39755=CARTESIAN_POINT('Ctrl Pts',(-21.2456232056939,18.7156729639725,-16.942021499332));
#39756=CARTESIAN_POINT('Ctrl Pts',(-21.263411741867,18.8058721596512,-16.946598776793));
#39757=CARTESIAN_POINT('Ctrl Pts',(-21.2763633328307,18.897163189666,-16.951176054254));
#39758=CARTESIAN_POINT('Ctrl Pts',(-21.2843593339857,18.9890376888929,-16.955753331715));
#39759=CARTESIAN_POINT('Ctrl Pts',(-21.2907392715853,19.0623435277363,-16.9594055003441));
#39760=CARTESIAN_POINT('Ctrl Pts',(-21.2939652250926,19.136020399912,-16.9630576689733));
#39761=CARTESIAN_POINT('Ctrl Pts',(-21.2939997202205,19.2098031412724,-16.9667098376024));
#39762=CARTESIAN_POINT('Origin',(-18.734,19.211,1.76670989022852));
#39763=CARTESIAN_POINT('',(-17.1721129955817,21.2441651167962,-15.6501589752972));
#39764=CARTESIAN_POINT('',(-17.1744642439897,21.2411350264762,-15.7166572006354));
#39765=CARTESIAN_POINT('',(-17.1744642439897,21.2411350264762,1.76670989022852));
#39766=CARTESIAN_POINT('',(-21.2939992944986,19.2129005700935,-16.2332901098004));
#39767=CARTESIAN_POINT('Ctrl Pts',(-17.1744642439897,21.2411350264762,-15.7166572006354));
#39768=CARTESIAN_POINT('Ctrl Pts',(-17.105540262146,21.1881880979566,-15.7209678899666));
#39769=CARTESIAN_POINT('Ctrl Pts',(-17.0393403283499,21.1317462119357,-15.7252785792978));
#39770=CARTESIAN_POINT('Ctrl Pts',(-16.9762229643503,21.0721340341153,-15.729589268629));
#39771=CARTESIAN_POINT('Ctrl Pts',(-16.9150839698182,21.0143903581622,-15.7337648424291));
#39772=CARTESIAN_POINT('Ctrl Pts',(-16.8568374435405,20.9536725741277,-15.7379404162292));
#39773=CARTESIAN_POINT('Ctrl Pts',(-16.8017703156805,20.8903118968895,-15.7421159900293));
#39774=CARTESIAN_POINT('Ctrl Pts',(-16.7440303488595,20.8238758297897,-15.7464942371261));
#39775=CARTESIAN_POINT('Ctrl Pts',(-16.6897865983678,20.7545342647742,-15.7508724842228));
#39776=CARTESIAN_POINT('Ctrl Pts',(-16.6393195365599,20.6827043711569,-15.7552507313195));
#39777=CARTESIAN_POINT('Ctrl Pts',(-16.588852474752,20.6108744775396,-15.7596289784163));
#39778=CARTESIAN_POINT('Ctrl Pts',(-16.5421623435021,20.5365567821694,-15.764007225513));
#39779=CARTESIAN_POINT('Ctrl Pts',(-16.499473974098,20.4601971179787,-15.7683854726097));
#39780=CARTESIAN_POINT('Ctrl Pts',(-16.458673348906,20.3872141935449,-15.7725701070028));
#39781=CARTESIAN_POINT('Ctrl Pts',(-16.4213761508429,20.3120944357929,-15.7767547413958));
#39782=CARTESIAN_POINT('Ctrl Pts',(-16.3878121523982,20.235208271674,-15.7809393757889));
#39783=CARTESIAN_POINT('Ctrl Pts',(-16.3542959281508,20.1584315454929,-15.7851180538728));
#39784=CARTESIAN_POINT('Ctrl Pts',(-16.3245025312235,20.0798938250627,-15.7892967319568));
#39785=CARTESIAN_POINT('Ctrl Pts',(-16.2986164546583,19.9999911197719,-15.7934754100407));
#39786=CARTESIAN_POINT('Ctrl Pts',(-16.2722663887748,19.918656215914,-15.7977289879262));
#39787=CARTESIAN_POINT('Ctrl Pts',(-16.2499653337518,19.8359073320096,-15.8019825658116));
#39788=CARTESIAN_POINT('Ctrl Pts',(-16.2318570828657,19.7521846470793,-15.806236143697));
#39789=CARTESIAN_POINT('Ctrl Pts',(-16.2140998957582,19.6700850897677,-15.810407257675));
#39790=CARTESIAN_POINT('Ctrl Pts',(-16.2003744938965,19.5870496228932,-15.8145783716529));
#39791=CARTESIAN_POINT('Ctrl Pts',(-16.1907660223745,19.5035080085245,-15.8187494856309));
#39792=CARTESIAN_POINT('Ctrl Pts',(-16.1811607750678,19.4199944273513,-15.8229191999512));
#39793=CARTESIAN_POINT('Ctrl Pts',(-16.1756697669882,19.3359754926339,-15.8270889142716));
#39794=CARTESIAN_POINT('Ctrl Pts',(-16.1743265551335,19.2518883314064,-15.831258628592));
#39795=CARTESIAN_POINT('Ctrl Pts',(-16.172983391076,19.167804162361,-15.835428194536));
#39796=CARTESIAN_POINT('Ctrl Pts',(-16.1757877362796,19.0836522316205,-15.8395977604801));
#39797=CARTESIAN_POINT('Ctrl Pts',(-16.1827210351531,18.9998705526709,-15.8437673264241));
#39798=CARTESIAN_POINT('Ctrl Pts',(-16.1898981002618,18.9131432132454,-15.848083489163));
#39799=CARTESIAN_POINT('Ctrl Pts',(-16.2014998257648,18.8268131717704,-15.8523996519019));
#39800=CARTESIAN_POINT('Ctrl Pts',(-16.2174472402026,18.7413594915726,-15.8567158146409));
#39801=CARTESIAN_POINT('Ctrl Pts',(-16.2328751692925,18.6586894560189,-15.8608913788325));
#39802=CARTESIAN_POINT('Ctrl Pts',(-16.2523698584566,18.5768400108849,-15.8650669430242));
#39803=CARTESIAN_POINT('Ctrl Pts',(-16.2758083142182,18.4962317606711,-15.8692425072159));
#39804=CARTESIAN_POINT('Ctrl Pts',(-16.3004305906606,18.4115521793672,-15.8736289692284));
#39805=CARTESIAN_POINT('Ctrl Pts',(-16.3294053113243,18.328243025166,-15.878015431241));
#39806=CARTESIAN_POINT('Ctrl Pts',(-16.3625325554083,18.2467686173736,-15.8824018932535));
#39807=CARTESIAN_POINT('Ctrl Pts',(-16.3956597994923,18.1652942095812,-15.886788355266));
#39808=CARTESIAN_POINT('Ctrl Pts',(-16.4329392521204,18.0856550414425,-15.8911748172785));
#39809=CARTESIAN_POINT('Ctrl Pts',(-16.4741163568262,18.0082839406928,-15.8955612792911));
#39810=CARTESIAN_POINT('Ctrl Pts',(-16.5133988419055,17.9344727989798,-15.8997459136841));
#39811=CARTESIAN_POINT('Ctrl Pts',(-16.5563744043013,17.8624508577059,-15.9039305480772));
#39812=CARTESIAN_POINT('Ctrl Pts',(-16.6028559450595,17.7926118242556,-15.9081151824702));
#39813=CARTESIAN_POINT('Ctrl Pts',(-16.6492713250977,17.722872198025,-15.9122938605542));
#39814=CARTESIAN_POINT('Ctrl Pts',(-16.6991825184353,17.6553096876334,-15.9164725386381));
#39815=CARTESIAN_POINT('Ctrl Pts',(-16.752356406431,17.5902937749033,-15.9206512167221));
#39816=CARTESIAN_POINT('Ctrl Pts',(-16.8064833981537,17.5241124986637,-15.9249047946075));
#39817=CARTESIAN_POINT('Ctrl Pts',(-16.8639909761116,17.460570439207,-15.9291583724929));
#39818=CARTESIAN_POINT('Ctrl Pts',(-16.9245868519813,17.400026764478,-15.9334119503784));
#39819=CARTESIAN_POINT('Ctrl Pts',(-16.9840079585542,17.3406568470249,-15.9375830643563));
#39820=CARTESIAN_POINT('Ctrl Pts',(-17.0463983458432,17.2841704328241,-15.9417541783343));
#39821=CARTESIAN_POINT('Ctrl Pts',(-17.1114427393843,17.2308717374818,-15.9459252923122));
#39822=CARTESIAN_POINT('Ctrl Pts',(-17.176465306651,17.1775909270316,-15.9500950066326));
#39823=CARTESIAN_POINT('Ctrl Pts',(-17.2441397559353,17.12749600239,-15.954264720953));
#39824=CARTESIAN_POINT('Ctrl Pts',(-17.3141166963449,17.0808517882548,-15.9584344352734));
#39825=CARTESIAN_POINT('Ctrl Pts',(-17.3840911466745,17.0342092339209,-15.9626040012174));
#39826=CARTESIAN_POINT('Ctrl Pts',(-17.4563675419654,16.9910174003976,-15.9667735671614));
#39827=CARTESIAN_POINT('Ctrl Pts',(-17.5305675384036,16.9514977737617,-15.9709431331055));
#39828=CARTESIAN_POINT('Ctrl Pts',(-17.6073763151811,16.9105886858059,-15.9752592958444));
#39829=CARTESIAN_POINT('Ctrl Pts',(-17.6862460120071,16.8736150868692,-15.9795754585833));
#39830=CARTESIAN_POINT('Ctrl Pts',(-17.7667310666841,16.8407698823443,-15.9838916213223));
#39831=CARTESIAN_POINT('Ctrl Pts',(-17.8445943291705,16.8089946069022,-15.9880671855139));
#39832=CARTESIAN_POINT('Ctrl Pts',(-17.923968865071,16.7810830031343,-15.9922427497056));
#39833=CARTESIAN_POINT('Ctrl Pts',(-18.0044344385269,16.7571593182294,-15.9964183138973));
#39834=CARTESIAN_POINT('Ctrl Pts',(-18.0889641368094,16.732027304873,-16.0008047759098));
#39835=CARTESIAN_POINT('Ctrl Pts',(-18.1746974182797,16.711296794516,-16.0051912379224));
#39836=CARTESIAN_POINT('Ctrl Pts',(-18.2611356505437,16.6950510126369,-16.0095776999349));
#39837=CARTESIAN_POINT('Ctrl Pts',(-18.3475738828078,16.6788052307578,-16.0139641619475));
#39838=CARTESIAN_POINT('Ctrl Pts',(-18.434716480688,16.6670441795795,-16.01835062396));
#39839=CARTESIAN_POINT('Ctrl Pts',(-18.5220617179684,16.6597880988421,-16.0227370859726));
#39840=CARTESIAN_POINT('Ctrl Pts',(-18.6053880714047,16.6528658811356,-16.0269217203656));
#39841=CARTESIAN_POINT('Ctrl Pts',(-18.6892089831255,16.6500174172729,-16.0311063547587));
#39842=CARTESIAN_POINT('Ctrl Pts',(-18.7730921344107,16.6512984929826,-16.0352909891517));
#39843=CARTESIAN_POINT('Ctrl Pts',(-18.856855888413,16.6525777452396,-16.0394696672357));
#39844=CARTESIAN_POINT('Ctrl Pts',(-18.9406812499664,16.6579748547684,-16.0436483453196));
#39845=CARTESIAN_POINT('Ctrl Pts',(-19.0241313606307,16.6674937991861,-16.0478270234036));
#39846=CARTESIAN_POINT('Ctrl Pts',(-19.1090772545541,16.6771833638415,-16.052080601289));
#39847=CARTESIAN_POINT('Ctrl Pts',(-19.1936338320393,16.6911440245191,-16.0563341791744));
#39848=CARTESIAN_POINT('Ctrl Pts',(-19.2773408795587,16.7093244237911,-16.0605877570599));
#39849=CARTESIAN_POINT('Ctrl Pts',(-19.359425102621,16.727152360547,-16.0647588710378));
#39850=CARTESIAN_POINT('Ctrl Pts',(-19.4406919711072,16.7490377781069,-16.0689299850158));
#39851=CARTESIAN_POINT('Ctrl Pts',(-19.5207150357479,16.7748802466775,-16.0731010989937));
#39852=CARTESIAN_POINT('Ctrl Pts',(-19.6007112478765,16.8007140435582,-16.0772708133141));
#39853=CARTESIAN_POINT('Ctrl Pts',(-19.6794640476567,16.8305021131095,-16.0814405276345));
#39854=CARTESIAN_POINT('Ctrl Pts',(-19.7565616407636,16.8640940174692,-16.0856102419549));
#39855=CARTESIAN_POINT('Ctrl Pts',(-19.8336564904072,16.8976847264848,-16.0897798078989));
#39856=CARTESIAN_POINT('Ctrl Pts',(-19.9090958290854,16.9350788166487,-16.093949373843));
#39857=CARTESIAN_POINT('Ctrl Pts',(-19.9824886317276,16.9760780469003,-16.098118939787));
#39858=CARTESIAN_POINT('Ctrl Pts',(-20.0584618347708,17.0185187595094,-16.1024351025259));
#39859=CARTESIAN_POINT('Ctrl Pts',(-20.1322414512874,17.0648225852953,-16.1067512652649));
#39860=CARTESIAN_POINT('Ctrl Pts',(-20.2034241040032,17.1147192929919,-16.1110674280038));
#39861=CARTESIAN_POINT('Ctrl Pts',(-20.272287989294,17.1629906206835,-16.1152429921955));
#39862=CARTESIAN_POINT('Ctrl Pts',(-20.3387211617817,17.2146240223492,-16.1194185563871));
#39863=CARTESIAN_POINT('Ctrl Pts',(-20.4023916835429,17.2693333987821,-16.1235941205788));
#39864=CARTESIAN_POINT('Ctrl Pts',(-20.4692780519958,17.3268060157594,-16.1279805825913));
#39865=CARTESIAN_POINT('Ctrl Pts',(-20.5331149297311,17.3876731058189,-16.1323670446039));
#39866=CARTESIAN_POINT('Ctrl Pts',(-20.5935624370344,17.4515604464004,-16.1367535066164));
#39867=CARTESIAN_POINT('Ctrl Pts',(-20.6540099443376,17.515447786982,-16.141139968629));
#39868=CARTESIAN_POINT('Ctrl Pts',(-20.7110677625942,17.5823548872471,-16.1455264306415));
#39869=CARTESIAN_POINT('Ctrl Pts',(-20.764447298501,17.6518708302357,-16.149912892654));
#39870=CARTESIAN_POINT('Ctrl Pts',(-20.8154455601759,17.7182856499018,-16.1541036735168));
#39871=CARTESIAN_POINT('Ctrl Pts',(-20.8632791399794,17.7873320135741,-16.1582944543796));
#39872=CARTESIAN_POINT('Ctrl Pts',(-20.9076654294934,17.8586765917041,-16.1624852352424));
#39873=CARTESIAN_POINT('Ctrl Pts',(-20.9519891627481,17.929920619642,-16.1666701097864));
#39874=CARTESIAN_POINT('Ctrl Pts',(-20.9928750133147,18.0034560458724,-16.1708549843304));
#39875=CARTESIAN_POINT('Ctrl Pts',(-21.0300812471761,18.0789174471947,-16.1750398588744));
#39876=CARTESIAN_POINT('Ctrl Pts',(-21.0672460755937,18.1542948703099,-16.1792200762261));
#39877=CARTESIAN_POINT('Ctrl Pts',(-21.1007392197539,18.2315936031769,-16.1834002935778));
#39878=CARTESIAN_POINT('Ctrl Pts',(-21.1303635397438,18.310421416318,-16.1875805109295));
#39879=CARTESIAN_POINT('Ctrl Pts',(-21.1599640139561,18.3891857778594,-16.1917573634602));
#39880=CARTESIAN_POINT('Ctrl Pts',(-21.1857016914127,18.4694763469324,-16.1959342159909));
#39881=CARTESIAN_POINT('Ctrl Pts',(-21.2074270380287,18.550879793107,-16.2001110685216));
#39882=CARTESIAN_POINT('Ctrl Pts',(-21.2291418983469,18.6322439478127,-16.2042859049869));
#39883=CARTESIAN_POINT('Ctrl Pts',(-21.2468481598048,18.7147194701813,-16.2084607414522));
#39884=CARTESIAN_POINT('Ctrl Pts',(-21.2604461548154,18.7978779516678,-16.2126355779175));
#39885=CARTESIAN_POINT('Ctrl Pts',(-21.2740449836496,18.881041532398,-16.2168106703821));
#39886=CARTESIAN_POINT('Ctrl Pts',(-21.2835349604935,18.9648877054714,-16.2209857628466));
#39887=CARTESIAN_POINT('Ctrl Pts',(-21.2888677421723,19.0489789519614,-16.2251608553112));
#39888=CARTESIAN_POINT('Ctrl Pts',(-21.2923288662564,19.1035565169218,-16.227870606798));
#39889=CARTESIAN_POINT('Ctrl Pts',(-21.2940398771788,19.1582371483247,-16.2305803582847));
#39890=CARTESIAN_POINT('Ctrl Pts',(-21.293999294499,19.2129005695107,-16.2332901097715));
#39891=CARTESIAN_POINT('Ctrl Pts',(-21.2939992944986,19.2129005700935,-16.2332901098004));
#39892=CARTESIAN_POINT('Ctrl Pts',(-21.2939272486892,19.3099436741152,-16.2381006886061));
#39893=CARTESIAN_POINT('Ctrl Pts',(-21.2883332378637,19.4067618611679,-16.2429112674118));
#39894=CARTESIAN_POINT('Ctrl Pts',(-21.2773175036261,19.5027808694022,-16.2477218462175));
#39895=CARTESIAN_POINT('Ctrl Pts',(-21.2661096544807,19.6004744535223,-16.2526163217372));
#39896=CARTESIAN_POINT('Ctrl Pts',(-21.2492893600036,19.6973405506026,-16.2575107972568));
#39897=CARTESIAN_POINT('Ctrl Pts',(-21.2270132516536,19.792794574639,-16.2624052727765));
#39898=CARTESIAN_POINT('Ctrl Pts',(-21.2047371433036,19.8882485986755,-16.2672997482961));
#39899=CARTESIAN_POINT('Ctrl Pts',(-21.1770053785922,19.9822904288902,-16.2721942238158));
#39900=CARTESIAN_POINT('Ctrl Pts',(-21.1440235064311,20.074357804418,-16.2770886993354));
#39901=CARTESIAN_POINT('Ctrl Pts',(-21.1158249638011,20.1530727360925,-16.2812733337285));
#39902=CARTESIAN_POINT('Ctrl Pts',(-21.0837134704203,20.2305511910393,-16.2854579681215));
#39903=CARTESIAN_POINT('Ctrl Pts',(-21.0478172393665,20.3063765484118,-16.2896426025146));
#39904=CARTESIAN_POINT('Ctrl Pts',(-21.0119721021545,20.3820939777732,-16.2938212805985));
#39905=CARTESIAN_POINT('Ctrl Pts',(-20.9723531229123,20.4561625710811,-16.2979999586825));
#39906=CARTESIAN_POINT('Ctrl Pts',(-20.9291375533232,20.5281830252437,-16.3021786367664));
#39907=CARTESIAN_POINT('Ctrl Pts',(-20.8851473757077,20.601494394287,-16.3064322146518));
#39908=CARTESIAN_POINT('Ctrl Pts',(-20.8374305643565,20.6726830222908,-16.3106857925373));
#39909=CARTESIAN_POINT('Ctrl Pts',(-20.7862244101177,20.7413512572338,-16.3149393704227));
#39910=CARTESIAN_POINT('Ctrl Pts',(-20.7360109870995,20.8086882244473,-16.3191104844007));
#39911=CARTESIAN_POINT('Ctrl Pts',(-20.6824425969519,20.873601266221,-16.3232815983786));
#39912=CARTESIAN_POINT('Ctrl Pts',(-20.6257872198946,20.9357437823176,-16.3274527123566));
#39913=CARTESIAN_POINT('Ctrl Pts',(-20.5691508540963,20.9978654458928,-16.331622426677));
#39914=CARTESIAN_POINT('Ctrl Pts',(-20.5094298683183,21.0572180904716,-16.3357921409973));
#39915=CARTESIAN_POINT('Ctrl Pts',(-20.4469316957122,21.1134891605011,-16.3399618553177));
#39916=CARTESIAN_POINT('Ctrl Pts',(-20.3844357470594,21.1697582281645,-16.3441314212617));
#39917=CARTESIAN_POINT('Ctrl Pts',(-20.3191631505145,21.2229456321213,-16.3483009872058));
#39918=CARTESIAN_POINT('Ctrl Pts',(-20.2514562536424,21.2727775142535,-16.3524705531498));
#39919=CARTESIAN_POINT('Ctrl Pts',(-20.1813688658018,21.3243614238873,-16.3567867158888));
#39920=CARTESIAN_POINT('Ctrl Pts',(-20.1086732374466,21.372349148503,-16.3611028786277));
#39921=CARTESIAN_POINT('Ctrl Pts',(-20.0337823603681,21.4164853923062,-16.3654190413666));
#39922=CARTESIAN_POINT('Ctrl Pts',(-19.9613310457333,21.4591839026097,-16.3695946055583));
#39923=CARTESIAN_POINT('Ctrl Pts',(-19.8868257455395,21.498277825633,-16.37377016975));
#39924=CARTESIAN_POINT('Ctrl Pts',(-19.8106643175712,21.5335834640049,-16.3779457339416));
#39925=CARTESIAN_POINT('Ctrl Pts',(-19.7306561569328,21.5706723062398,-16.3823321959542));
#39926=CARTESIAN_POINT('Ctrl Pts',(-19.6488207114389,21.6035798961264,-16.3867186579667));
#39927=CARTESIAN_POINT('Ctrl Pts',(-19.565639342473,21.6321517928562,-16.3911051199793));
#39928=CARTESIAN_POINT('Ctrl Pts',(-19.4824579735071,21.6607236895861,-16.3954915819918));
#39929=CARTESIAN_POINT('Ctrl Pts',(-19.3979312597773,21.6849598063577,-16.3998780440043));
#39930=CARTESIAN_POINT('Ctrl Pts',(-19.3125527301391,21.7047675790756,-16.4042645060169));
#39931=CARTESIAN_POINT('Ctrl Pts',(-19.2310959760761,21.7236655019802,-16.4084494803761));
#39932=CARTESIAN_POINT('Ctrl Pts',(-19.1485607217984,21.7386033270999,-16.4126344547353));
#39933=CARTESIAN_POINT('Ctrl Pts',(-19.0653667817849,21.7494633257011,-16.4168194290945));
#39934=CARTESIAN_POINT('Ctrl Pts',(-18.9823149545843,21.760304773132,-16.420997254634));
#39935=CARTESIAN_POINT('Ctrl Pts',(-18.8986071312342,21.767082185981,-16.4251750801735));
#39936=CARTESIAN_POINT('Ctrl Pts',(-18.8146747410986,21.7697285096603,-16.4293529057129));
#39937=CARTESIAN_POINT('Ctrl Pts',(-18.7308239310027,21.7723722611837,-16.4335266705177));
#39938=CARTESIAN_POINT('Ctrl Pts',(-18.6467494445132,21.7708928806729,-16.4377004353224));
#39939=CARTESIAN_POINT('Ctrl Pts',(-18.5628884909282,21.7652750148453,-16.4418742001271));
#39940=CARTESIAN_POINT('Ctrl Pts',(-18.4790838891784,21.759660924041,-16.4460451602976));
#39941=CARTESIAN_POINT('Ctrl Pts',(-18.395492992995,21.7499139014376,-16.450216120468));
#39942=CARTESIAN_POINT('Ctrl Pts',(-18.3125523069991,21.7360706608062,-16.4543870806384));
#39943=CARTESIAN_POINT('Ctrl Pts',(-18.2296424734748,21.722232569616,-16.4585564892853));
#39944=CARTESIAN_POINT('Ctrl Pts',(-18.147382822705,21.7043013640785,-16.4627258979321));
#39945=CARTESIAN_POINT('Ctrl Pts',(-18.0662026746013,21.6823653578923,-16.466895306579));
#39946=CARTESIAN_POINT('Ctrl Pts',(-17.9849897282951,21.6604204891752,-16.47106639974));
#39947=CARTESIAN_POINT('Ctrl Pts',(-17.904857603049,21.6344676983622,-16.475237492901));
#39948=CARTESIAN_POINT('Ctrl Pts',(-17.826222656682,21.6046458165231,-16.479408586062));
#39949=CARTESIAN_POINT('Ctrl Pts',(-17.747575565893,21.5748193289771,-16.4835803234088));
#39950=CARTESIAN_POINT('Ctrl Pts',(-17.670426540659,21.5411227351731,-16.4877520607556));
#39951=CARTESIAN_POINT('Ctrl Pts',(-17.5951721111185,21.5037431254953,-16.4919237981024));
#39952=CARTESIAN_POINT('Ctrl Pts',(-17.5198228509081,21.466316412498,-16.4961007923975));
#39953=CARTESIAN_POINT('Ctrl Pts',(-17.4463733641076,21.4251976266706,-16.5002777866927));
#39954=CARTESIAN_POINT('Ctrl Pts',(-17.3751954108584,21.3806198027598,-16.5044547809878));
#39955=CARTESIAN_POINT('Ctrl Pts',(-17.3060362702805,21.3373063348984,-16.5085133036407));
#39956=CARTESIAN_POINT('Ctrl Pts',(-17.2390218174128,21.2907277100965,-16.5125718262936));
#39957=CARTESIAN_POINT('Ctrl Pts',(-17.1744642439897,21.2411350264762,-16.5166303489465));
#39958=CARTESIAN_POINT('',(-21.2939994369002,19.2093020392337,-16.1667098902285));
#39959=CARTESIAN_POINT('Ctrl Pts',(-21.2939994369002,19.2093020392337,-16.1667098902285));
#39960=CARTESIAN_POINT('Ctrl Pts',(-21.2940542005915,19.2918687402816,-16.1708335669039));
#39961=CARTESIAN_POINT('Ctrl Pts',(-21.2901102644712,19.37459277435,-16.1749572435793));
#39962=CARTESIAN_POINT('Ctrl Pts',(-21.282148407848,19.4570481489096,-16.1790809202548));
#39963=CARTESIAN_POINT('Ctrl Pts',(-21.2741500199359,19.5398818524497,-16.1832235175451));
#39964=CARTESIAN_POINT('Ctrl Pts',(-21.2620966823448,19.6224439445467,-16.1873661148355));
#39965=CARTESIAN_POINT('Ctrl Pts',(-21.2460219433305,19.7043008779902,-16.1915087121259));
#39966=CARTESIAN_POINT('Ctrl Pts',(-21.23005430851,19.7856124078128,-16.1956237077524));
#39967=CARTESIAN_POINT('Ctrl Pts',(-21.2101187777554,19.8662276743518,-16.1997387033789));
#39968=CARTESIAN_POINT('Ctrl Pts',(-21.1863001253011,19.9457272251988,-16.2038536990054));
#39969=CARTESIAN_POINT('Ctrl Pts',(-21.1624916905597,20.0251926723701,-16.2079669293832));
#39970=CARTESIAN_POINT('Ctrl Pts',(-21.13480357533,20.1035429002386,-16.2120801597611));
#39971=CARTESIAN_POINT('Ctrl Pts',(-21.1033710027996,20.1803714721883,-16.2161933901389));
#39972=CARTESIAN_POINT('Ctrl Pts',(-21.0719418753925,20.2571916234494,-16.2203061696919));
#39973=CARTESIAN_POINT('Ctrl Pts',(-21.0367692860285,20.3324900117991,-16.2244189492448));
#39974=CARTESIAN_POINT('Ctrl Pts',(-20.998036835518,20.405879578626,-16.2285317287978));
#39975=CARTESIAN_POINT('Ctrl Pts',(-20.9588192445656,20.48018838104,-16.2326960226666));
#39976=CARTESIAN_POINT('Ctrl Pts',(-20.9159522062818,20.5525397612551,-16.2368603165354));
#39977=CARTESIAN_POINT('Ctrl Pts',(-20.8696736494983,20.6225587351713,-16.2410246104042));
#39978=CARTESIAN_POINT('Ctrl Pts',(-20.8239074514183,20.6918025157111,-16.2451428005837));
#39979=CARTESIAN_POINT('Ctrl Pts',(-20.7748052350545,20.7587649302322,-16.2492609907631));
#39980=CARTESIAN_POINT('Ctrl Pts',(-20.7226388747276,20.823115202435,-16.2533791809425));
#39981=CARTESIAN_POINT('Ctrl Pts',(-20.6695965003383,20.8885460894827,-16.257566526656));
#39982=CARTESIAN_POINT('Ctrl Pts',(-20.6133864683218,20.9512759179512,-16.2617538723695));
#39983=CARTESIAN_POINT('Ctrl Pts',(-20.5543334369044,21.0109961606869,-16.265941218083));
#39984=CARTESIAN_POINT('Ctrl Pts',(-20.495280405487,21.0707164034227,-16.2701285637965));
#39985=CARTESIAN_POINT('Ctrl Pts',(-20.4333847973435,21.1274267716985,-16.2743159095101));
#39986=CARTESIAN_POINT('Ctrl Pts',(-20.369004471075,21.1808630357374,-16.2785032552236));
#39987=CARTESIAN_POINT('Ctrl Pts',(-20.3046658312849,21.2342646996152,-16.2826878896166));
#39988=CARTESIAN_POINT('Ctrl Pts',(-20.2375884427955,21.2846103343966,-16.2868725240096));
#39989=CARTESIAN_POINT('Ctrl Pts',(-20.1680947292201,21.3316065895453,-16.2910571584027));
#39990=CARTESIAN_POINT('Ctrl Pts',(-20.0986999313442,21.378535951342,-16.2952358364866));
#39991=CARTESIAN_POINT('Ctrl Pts',(-20.0268960178075,21.4221251476138,-16.2994145145706));
#39992=CARTESIAN_POINT('Ctrl Pts',(-19.9530388079931,21.4621206952553,-16.3035931926545));
#39993=CARTESIAN_POINT('Ctrl Pts',(-19.877857760773,21.502833134344,-16.30784677054));
#39994=CARTESIAN_POINT('Ctrl Pts',(-19.800549453568,21.5398215173808,-16.3121003484254));
#39995=CARTESIAN_POINT('Ctrl Pts',(-19.7215205448428,21.5728643427414,-16.3163539263108));
#39996=CARTESIAN_POINT('Ctrl Pts',(-19.6440237657254,21.6052665684547,-16.3205250402888));
#39997=CARTESIAN_POINT('Ctrl Pts',(-19.5648729481498,21.6338746703222,-16.3246961542667));
#39998=CARTESIAN_POINT('Ctrl Pts',(-19.4844751811847,21.6585267112793,-16.3288672682447));
#39999=CARTESIAN_POINT('Ctrl Pts',(-19.4041043924667,21.683170480006,-16.3330369825651));
#40000=CARTESIAN_POINT('Ctrl Pts',(-19.3224879248151,21.7038606894987,-16.3372066968855));
#40001=CARTESIAN_POINT('Ctrl Pts',(-19.2400494979668,21.7204847888775,-16.3413764112058));
#40002=CARTESIAN_POINT('Ctrl Pts',(-19.1576140046316,21.7371082966994,-16.3455459771499));
#40003=CARTESIAN_POINT('Ctrl Pts',(-19.0743570613777,21.7496658919856,-16.3497155430939));
#40004=CARTESIAN_POINT('Ctrl Pts',(-18.9907127437439,21.758096104822,-16.3538851090379));
#40005=CARTESIAN_POINT('Ctrl Pts',(-18.9041275950885,21.7668227135419,-16.3582012717769));
#40006=CARTESIAN_POINT('Ctrl Pts',(-18.8171278498233,21.7711262492444,-16.3625174345158));
#40007=CARTESIAN_POINT('Ctrl Pts',(-18.7301989430818,21.7709971781169,-16.3668335972547));
#40008=CARTESIAN_POINT('Ctrl Pts',(-18.646101736334,21.7708723114677,-16.3710091614464));
#40009=CARTESIAN_POINT('Ctrl Pts',(-18.5620712918898,21.7665992585964,-16.3751847256381));
#40010=CARTESIAN_POINT('Ctrl Pts',(-18.478543574057,21.7582224116563,-16.3793602898297));
#40011=CARTESIAN_POINT('Ctrl Pts',(-18.3907970697647,21.7494224700914,-16.3837467518423));
#40012=CARTESIAN_POINT('Ctrl Pts',(-18.3036059893692,21.7360933624401,-16.3881332138548));
#40013=CARTESIAN_POINT('Ctrl Pts',(-18.2174632822105,21.7183471676605,-16.3925196758674));
#40014=CARTESIAN_POINT('Ctrl Pts',(-18.1313205750519,21.700600972881,-16.3969061378799));
#40015=CARTESIAN_POINT('Ctrl Pts',(-18.0462267834431,21.6784379108237,-16.4012925998925));
#40016=CARTESIAN_POINT('Ctrl Pts',(-17.9626538344088,21.652029514944,-16.405679061905));
#40017=CARTESIAN_POINT('Ctrl Pts',(-17.8829440436939,21.6268418467689,-16.4098627597766));
#40018=CARTESIAN_POINT('Ctrl Pts',(-17.804320970107,21.5976989266328,-16.4140464576482));
#40019=CARTESIAN_POINT('Ctrl Pts',(-17.7272055153236,21.5647129955934,-16.4182301555198));
#40020=CARTESIAN_POINT('Ctrl Pts',(-17.6501861872981,21.5317681825194,-16.4224086382849));
#40021=CARTESIAN_POINT('Ctrl Pts',(-17.5746711676834,21.4949900441651,-16.42658712105));
#40022=CARTESIAN_POINT('Ctrl Pts',(-17.501066141267,21.4545405278242,-16.430765603815));
#40023=CARTESIAN_POINT('Ctrl Pts',(-17.4275438124869,21.4141364578278,-16.4349393919191));
#40024=CARTESIAN_POINT('Ctrl Pts',(-17.3559276132931,21.3700694275063,-16.4391131800231));
#40025=CARTESIAN_POINT('Ctrl Pts',(-17.286601701979,21.3225487602435,-16.4432869681272));
#40026=CARTESIAN_POINT('Ctrl Pts',(-17.2485114006814,21.2964390921614,-16.445580206592));
#40027=CARTESIAN_POINT('Ctrl Pts',(-17.2111121045273,21.2692876607317,-16.4478734450569));
#40028=CARTESIAN_POINT('Ctrl Pts',(-17.1744642439897,21.2411350264762,-16.4501666835217));
#40029=CARTESIAN_POINT('Ctrl Pts',(-17.1721129955817,21.2441651167962,-15.6501589752972));
#40030=CARTESIAN_POINT('Ctrl Pts',(-16.5413044024314,20.7545799890971,-15.6900393263641));
#40031=CARTESIAN_POINT('Ctrl Pts',(-15.7364333696473,19.087953254603,-15.7723116129914));
#40032=CARTESIAN_POINT('Ctrl Pts',(-17.157742779603,16.6266809758552,-15.8969758351793));
#40033=CARTESIAN_POINT('Ctrl Pts',(-20.0538051846353,16.4867742534768,-16.0241516418607));
#40034=CARTESIAN_POINT('Ctrl Pts',(-21.2452321357866,18.1548349245933,-16.1140629935438));
#40035=CARTESIAN_POINT('Ctrl Pts',(-21.2975540665632,19.1065231701483,-16.1615824096664));
#40036=CARTESIAN_POINT('Ctrl Pts',(-21.2967674646518,19.2093002032948,-16.1667098902285));
#40037=CARTESIAN_POINT('Origin',(-18.734,19.211,1.76670989022852));
#40038=CARTESIAN_POINT('',(-17.1744642439897,21.2411350264762,-14.8500370213226));
#40039=CARTESIAN_POINT('',(-17.1744642439897,21.2411350264762,-14.9167585741126));
#40040=CARTESIAN_POINT('',(-17.1744642439897,21.2411350264762,1.76670989022852));
#40041=CARTESIAN_POINT('',(-21.293999428374,19.2092892327452,-15.4332901097416));
#40042=CARTESIAN_POINT('Ctrl Pts',(-17.1744642439897,21.2411350264762,-14.9167585741126));
#40043=CARTESIAN_POINT('Ctrl Pts',(-17.1078481116885,21.1899609720926,-14.9209295684745));
#40044=CARTESIAN_POINT('Ctrl Pts',(-17.043705379627,21.1354676782673,-14.9251005628365));
#40045=CARTESIAN_POINT('Ctrl Pts',(-16.9823784647263,21.0779284927831,-14.9292715571984));
#40046=CARTESIAN_POINT('Ctrl Pts',(-16.9210710217901,21.020407576618,-14.9334412272241));
#40047=CARTESIAN_POINT('Ctrl Pts',(-16.8625779555852,20.9598430040762,-14.9376108972499));
#40048=CARTESIAN_POINT('Ctrl Pts',(-16.8072070152721,20.8965470310861,-14.9417805672756));
#40049=CARTESIAN_POINT('Ctrl Pts',(-16.7518370459354,20.8332521680447,-14.9459501641826));
#40050=CARTESIAN_POINT('Ctrl Pts',(-16.6995893957288,20.7672263467399,-14.9501197610897));
#40051=CARTESIAN_POINT('Ctrl Pts',(-16.6507325669181,20.69881611843,-14.9542893579967));
#40052=CARTESIAN_POINT('Ctrl Pts',(-16.6008933205169,20.6290302909808,-14.9585427975404));
#40053=CARTESIAN_POINT('Ctrl Pts',(-16.5545830529723,20.5567635132021,-14.9627962370841));
#40054=CARTESIAN_POINT('Ctrl Pts',(-16.5120402532923,20.4824145209217,-14.9670496766278));
#40055=CARTESIAN_POINT('Ctrl Pts',(-16.4702752492726,20.4094248261953,-14.9712253519706));
#40056=CARTESIAN_POINT('Ctrl Pts',(-16.4321412641796,20.3344288611474,-14.9754010273135));
#40057=CARTESIAN_POINT('Ctrl Pts',(-16.3978164930544,20.2578269302399,-14.9795767026564));
#40058=CARTESIAN_POINT('Ctrl Pts',(-16.3625328692254,20.1790851462127,-14.9838690243005));
#40059=CARTESIAN_POINT('Ctrl Pts',(-16.3312746389474,20.0986468241009,-14.9881613459446));
#40060=CARTESIAN_POINT('Ctrl Pts',(-16.3041808829601,20.0169646756945,-14.9924536675887));
#40061=CARTESIAN_POINT('Ctrl Pts',(-16.2770871269728,19.9352825272881,-14.9967459892329));
#40062=CARTESIAN_POINT('Ctrl Pts',(-16.254157917113,19.8523570726247,-15.001038310877));
#40063=CARTESIAN_POINT('Ctrl Pts',(-16.2354754819719,19.7686515334978,-15.0053306325211));
#40064=CARTESIAN_POINT('Ctrl Pts',(-16.2172617582301,19.6870460279087,-15.0095152669141));
#40065=CARTESIAN_POINT('Ctrl Pts',(-16.2030163785017,19.6043953888035,-15.0136999013072));
#40066=CARTESIAN_POINT('Ctrl Pts',(-16.1928535263698,19.5211202985238,-15.0178845357002));
#40067=CARTESIAN_POINT('Ctrl Pts',(-16.1827051397999,19.4379637400279,-15.0220632137842));
#40068=CARTESIAN_POINT('Ctrl Pts',(-16.1766277936582,19.3541849485908,-15.0262418918681));
#40069=CARTESIAN_POINT('Ctrl Pts',(-16.1746849654928,19.2702161645613,-15.0304205699521));
#40070=CARTESIAN_POINT('Ctrl Pts',(-16.1727073135288,19.1847423004251,-15.0346741478375));
#40071=CARTESIAN_POINT('Ctrl Pts',(-16.1750139649456,19.0990720360283,-15.0389277257229));
#40072=CARTESIAN_POINT('Ctrl Pts',(-16.1816167614736,19.0136682902081,-15.0431813036084));
#40073=CARTESIAN_POINT('Ctrl Pts',(-16.1880915499065,18.9299202626523,-15.0473524175863));
#40074=CARTESIAN_POINT('Ctrl Pts',(-16.1986973545604,18.8464289917134,-15.0515235315643));
#40075=CARTESIAN_POINT('Ctrl Pts',(-16.2133928011125,18.7636306348036,-15.0556946455422));
#40076=CARTESIAN_POINT('Ctrl Pts',(-16.2280833164655,18.6808600616823,-15.0598643598626));
#40077=CARTESIAN_POINT('Ctrl Pts',(-16.2468606679443,18.5987823933906,-15.064034074183));
#40078=CARTESIAN_POINT('Ctrl Pts',(-16.2696319425034,18.517826084456,-15.0682037885033));
#40079=CARTESIAN_POINT('Ctrl Pts',(-16.292402406763,18.4368726562941,-15.0723733544474));
#40080=CARTESIAN_POINT('Ctrl Pts',(-16.3191663861462,18.3570409507695,-15.0765429203914));
#40081=CARTESIAN_POINT('Ctrl Pts',(-16.3497807798975,18.278745361774,-15.0807124863355));
#40082=CARTESIAN_POINT('Ctrl Pts',(-16.3814715379662,18.1976969964576,-15.0850286490744));
#40083=CARTESIAN_POINT('Ctrl Pts',(-16.4172883172412,18.1182952684026,-15.0893448118133));
#40084=CARTESIAN_POINT('Ctrl Pts',(-16.4570183818635,18.040976619606,-15.0936609745523));
#40085=CARTESIAN_POINT('Ctrl Pts',(-16.4954542438097,17.9661766176614,-15.0978365387439));
#40086=CARTESIAN_POINT('Ctrl Pts',(-16.5375520792277,17.893326450692,-15.1020121029356));
#40087=CARTESIAN_POINT('Ctrl Pts',(-16.5830736962919,17.8227939504466,-15.1061876671273));
#40088=CARTESIAN_POINT('Ctrl Pts',(-16.6308945020167,17.7486990212889,-15.1105741291398));
#40089=CARTESIAN_POINT('Ctrl Pts',(-16.6824937078807,17.6771625161639,-15.1149605911524));
#40090=CARTESIAN_POINT('Ctrl Pts',(-16.7375469032624,17.6085721443613,-15.1193470531649));
#40091=CARTESIAN_POINT('Ctrl Pts',(-16.7926000986442,17.5399817725586,-15.1237335151774));
#40092=CARTESIAN_POINT('Ctrl Pts',(-16.851106840707,17.4743379166139,-15.12811997719));
#40093=CARTESIAN_POINT('Ctrl Pts',(-16.9126993772537,17.4119824788001,-15.1325064392025));
#40094=CARTESIAN_POINT('Ctrl Pts',(-16.971457949892,17.352496107113,-15.1366910735956));
#40095=CARTESIAN_POINT('Ctrl Pts',(-17.0332433037703,17.2957807737874,-15.1408757079886));
#40096=CARTESIAN_POINT('Ctrl Pts',(-17.0977635170214,17.2421601965193,-15.1450603423817));
#40097=CARTESIAN_POINT('Ctrl Pts',(-17.1621918937349,17.1886159415061,-15.1492390204656));
#40098=CARTESIAN_POINT('Ctrl Pts',(-17.2293470468518,17.1381579843473,-15.1534176985496));
#40099=CARTESIAN_POINT('Ctrl Pts',(-17.2988998898353,17.0910736631182,-15.1575963766335));
#40100=CARTESIAN_POINT('Ctrl Pts',(-17.3696994175425,17.0431453892699,-15.1618499545189));
#40101=CARTESIAN_POINT('Ctrl Pts',(-17.4429830989498,16.998713228823,-15.1661035324044));
#40102=CARTESIAN_POINT('Ctrl Pts',(-17.5183681022774,16.9580377079855,-15.1703571102898));
#40103=CARTESIAN_POINT('Ctrl Pts',(-17.5922916202138,16.9181507614911,-15.1745282242678));
#40104=CARTESIAN_POINT('Ctrl Pts',(-17.6682352871974,16.881876323378,-15.1786993382457));
#40105=CARTESIAN_POINT('Ctrl Pts',(-17.7458099687319,16.8494156881233,-15.1828704522237));
#40106=CARTESIAN_POINT('Ctrl Pts',(-17.8233586193327,16.8169659453482,-15.187040166544));
#40107=CARTESIAN_POINT('Ctrl Pts',(-17.9025367735083,16.7883276412413,-15.1912098808644));
#40108=CARTESIAN_POINT('Ctrl Pts',(-17.9829338767361,16.7636545649448,-15.1953795951848));
#40109=CARTESIAN_POINT('Ctrl Pts',(-18.0633281190899,16.7389823666223,-15.1995491611288));
#40110=CARTESIAN_POINT('Ctrl Pts',(-18.1449407842156,16.7182752497196,-15.2037187270729));
#40111=CARTESIAN_POINT('Ctrl Pts',(-18.2273459747046,16.7016371927017,-15.2078882930169));
#40112=CARTESIAN_POINT('Ctrl Pts',(-18.3126484300336,16.6844141621243,-15.2122044557558));
#40113=CARTESIAN_POINT('Ctrl Pts',(-18.3987996610347,16.671551755943,-15.2165206184947));
#40114=CARTESIAN_POINT('Ctrl Pts',(-18.485317539171,16.6631073347419,-15.2208367812337));
#40115=CARTESIAN_POINT('Ctrl Pts',(-18.5690171065272,16.6549379896732,-15.2250123454254));
#40116=CARTESIAN_POINT('Ctrl Pts',(-18.6530593280227,16.650903193465,-15.229187909617));
#40117=CARTESIAN_POINT('Ctrl Pts',(-18.7370059866502,16.6510017648357,-15.2333634738087));
#40118=CARTESIAN_POINT('Ctrl Pts',(-18.8251925914406,16.6511053148121,-15.2377499358213));
#40119=CARTESIAN_POINT('Ctrl Pts',(-18.9132731428314,16.6557707277653,-15.2421363978338));
#40120=CARTESIAN_POINT('Ctrl Pts',(-19.0007460413496,16.6649350853868,-15.2465228598464));
#40121=CARTESIAN_POINT('Ctrl Pts',(-19.0882189398677,16.6740994430083,-15.2509093218589));
#40122=CARTESIAN_POINT('Ctrl Pts',(-19.1750836241624,16.6877625800018,-15.2552957838714));
#40123=CARTESIAN_POINT('Ctrl Pts',(-19.2608535512398,16.7058003401833,-15.259682245884));
#40124=CARTESIAN_POINT('Ctrl Pts',(-19.3426770768309,16.7230081562804,-15.263866880277));
#40125=CARTESIAN_POINT('Ctrl Pts',(-19.4238089369641,16.74426092691,-15.2680515146701));
#40126=CARTESIAN_POINT('Ctrl Pts',(-19.5038189245164,16.7694884142285,-15.2722361490631));
#40127=CARTESIAN_POINT('Ctrl Pts',(-19.5837150277545,16.7946799933413,-15.2764148271471));
#40128=CARTESIAN_POINT('Ctrl Pts',(-19.662491995264,16.82383491438,-15.280593505231));
#40129=CARTESIAN_POINT('Ctrl Pts',(-19.7397300928951,16.8568319982964,-15.2847721833149));
#40130=CARTESIAN_POINT('Ctrl Pts',(-19.8183526279165,16.8904205312276,-15.2890257612004));
#40131=CARTESIAN_POINT('Ctrl Pts',(-19.8953801101213,16.9279902241697,-15.2932793390858));
#40132=CARTESIAN_POINT('Ctrl Pts',(-19.9703862586165,16.9693601940757,-15.2975329169713));
#40133=CARTESIAN_POINT('Ctrl Pts',(-20.0439382665606,17.0099281263882,-15.3017040309492));
#40134=CARTESIAN_POINT('Ctrl Pts',(-20.1155461950119,17.0541500666239,-15.3058751449272));
#40135=CARTESIAN_POINT('Ctrl Pts',(-20.1848301560486,17.1018077711361,-15.3100462589051));
#40136=CARTESIAN_POINT('Ctrl Pts',(-20.2540908681831,17.1494494836452,-15.3142159732255));
#40137=CARTESIAN_POINT('Ctrl Pts',(-20.3210287829499,17.2005244102477,-15.3183856875458));
#40138=CARTESIAN_POINT('Ctrl Pts',(-20.3852923626418,17.2547705827075,-15.3225554018662));
#40139=CARTESIAN_POINT('Ctrl Pts',(-20.4495536555597,17.3090148248555,-15.3267249678102));
#40140=CARTESIAN_POINT('Ctrl Pts',(-20.5111404516285,17.3664297911041,-15.3308945337543));
#40141=CARTESIAN_POINT('Ctrl Pts',(-20.5697347912246,17.4267136507031,-15.3350640996983));
#40142=CARTESIAN_POINT('Ctrl Pts',(-20.6303892355173,17.4891170164376,-15.3393802624373));
#40143=CARTESIAN_POINT('Ctrl Pts',(-20.6878365109494,17.5545943914706,-15.3436964251762));
#40144=CARTESIAN_POINT('Ctrl Pts',(-20.7417674193149,17.6227714301973,-15.3480125879151));
#40145=CARTESIAN_POINT('Ctrl Pts',(-20.7939415340127,17.6887276090582,-15.3521881521068));
#40146=CARTESIAN_POINT('Ctrl Pts',(-20.8428246196122,17.7572098587043,-15.3563637162985));
#40147=CARTESIAN_POINT('Ctrl Pts',(-20.8881804708293,17.8278490685766,-15.3605392804901));
#40148=CARTESIAN_POINT('Ctrl Pts',(-20.9358271382683,17.902056097011,-15.3649257425027));
#40149=CARTESIAN_POINT('Ctrl Pts',(-20.9795805961805,17.9786432012264,-15.3693122045152));
#40150=CARTESIAN_POINT('Ctrl Pts',(-21.0192222426251,18.0571545589588,-15.3736986665278));
#40151=CARTESIAN_POINT('Ctrl Pts',(-21.0588638890696,18.1356659166911,-15.3780851285404));
#40152=CARTESIAN_POINT('Ctrl Pts',(-21.0943935591861,18.2161009664615,-15.3824715905529));
#40153=CARTESIAN_POINT('Ctrl Pts',(-21.1256522921828,18.2979833992217,-15.3868580525655));
#40154=CARTESIAN_POINT('Ctrl Pts',(-21.1596866697224,18.3871366489942,-15.3916340140292));
#40155=CARTESIAN_POINT('Ctrl Pts',(-21.188765023978,18.4782809296074,-15.396409975493));
#40156=CARTESIAN_POINT('Ctrl Pts',(-21.2126811308611,18.5708907503299,-15.4011859369568));
#40157=CARTESIAN_POINT('Ctrl Pts',(-21.236499376369,18.6631216245769,-15.4059423558521));
#40158=CARTESIAN_POINT('Ctrl Pts',(-21.2551974088383,18.7568058878157,-15.4106987747474));
#40159=CARTESIAN_POINT('Ctrl Pts',(-21.2686182636666,18.8514026453274,-15.4154551936427));
#40160=CARTESIAN_POINT('Ctrl Pts',(-21.2819450244393,18.9453361818536,-15.4201782651283));
#40161=CARTESIAN_POINT('Ctrl Pts',(-21.2900682365864,19.0401692636774,-15.4249013366139));
#40162=CARTESIAN_POINT('Ctrl Pts',(-21.2928821031966,19.1353535728531,-15.4296244080995));
#40163=CARTESIAN_POINT('Ctrl Pts',(-21.2936100754836,19.1599785991387,-15.4308463086469));
#40164=CARTESIAN_POINT('Ctrl Pts',(-21.2939829474075,19.1846270439602,-15.4320682091942));
#40165=CARTESIAN_POINT('Ctrl Pts',(-21.293999428374,19.2092892327452,-15.4332901097416));
#40166=CARTESIAN_POINT('Ctrl Pts',(-21.2939994283744,19.2092892333484,-15.4332901097715));
#40167=CARTESIAN_POINT('Ctrl Pts',(-21.2940559692553,19.2938972788889,-15.437482057942));
#40168=CARTESIAN_POINT('Ctrl Pts',(-21.2899137324165,19.3785303101354,-15.4416740061124));
#40169=CARTESIAN_POINT('Ctrl Pts',(-21.2815918669692,19.4627452667924,-15.4458659542829));
#40170=CARTESIAN_POINT('Ctrl Pts',(-21.2732695913204,19.546964374574,-15.4500581090829));
#40171=CARTESIAN_POINT('Ctrl Pts',(-21.2607673227297,19.6307649161162,-15.4542502638829));
#40172=CARTESIAN_POINT('Ctrl Pts',(-21.2441560631152,19.7137091990464,-15.4584424186829));
#40173=CARTESIAN_POINT('Ctrl Pts',(-21.2275392030058,19.7966814466854,-15.4626359868702));
#40174=CARTESIAN_POINT('Ctrl Pts',(-21.2068106889623,19.878796418332,-15.4668295550574));
#40175=CARTESIAN_POINT('Ctrl Pts',(-21.1820923104738,19.9596281048684,-15.4710231232446));
#40176=CARTESIAN_POINT('Ctrl Pts',(-21.157341575289,20.0405656011908,-15.4752221808701));
#40177=CARTESIAN_POINT('Ctrl Pts',(-21.1285906849039,20.1202160261787,-15.4794212384956));
#40178=CARTESIAN_POINT('Ctrl Pts',(-21.0960107310932,20.1981703531815,-15.483620296121));
#40179=CARTESIAN_POINT('Ctrl Pts',(-21.0634063961448,20.2761830171356,-15.4878224961022));
#40180=CARTESIAN_POINT('Ctrl Pts',(-21.0269674888695,20.3524966484648,-15.4920246960833));
#40181=CARTESIAN_POINT('Ctrl Pts',(-20.9869114421225,20.4267261344371,-15.4962268960644));
#40182=CARTESIAN_POINT('Ctrl Pts',(-20.9467843119665,20.5010873479597,-15.5004365532642));
#40183=CARTESIAN_POINT('Ctrl Pts',(-20.903027463882,20.5733566470828,-15.504646210464));
#40184=CARTESIAN_POINT('Ctrl Pts',(-20.8559018807143,20.6431775059751,-15.5088558676638));
#40185=CARTESIAN_POINT('Ctrl Pts',(-20.8365799691026,20.6718046841124,-15.5105818648582));
#40186=CARTESIAN_POINT('Ctrl Pts',(-20.8166922183619,20.7000206489315,-15.5123078620525));
#40187=CARTESIAN_POINT('Ctrl Pts',(-20.7962584977301,20.7278025212729,-15.5140338592469));
#40188=CARTESIAN_POINT('Ctrl Pts',(-20.7467174843304,20.7951589334867,-15.5182184936399));
#40189=CARTESIAN_POINT('Ctrl Pts',(-20.6937808669813,20.8602110167103,-15.522403128033));
#40190=CARTESIAN_POINT('Ctrl Pts',(-20.6376906991395,20.9225962497066,-15.526587762426));
#40191=CARTESIAN_POINT('Ctrl Pts',(-20.5816803687091,20.9848926850455,-15.53076644051));
#40192=CARTESIAN_POINT('Ctrl Pts',(-20.5225257086781,21.0445294709031,-15.5349451185939));
#40193=CARTESIAN_POINT('Ctrl Pts',(-20.4605108062945,21.1011747103769,-15.5391237966779));
#40194=CARTESIAN_POINT('Ctrl Pts',(-20.397384331355,21.158835275058,-15.5433773745633));
#40195=CARTESIAN_POINT('Ctrl Pts',(-20.3312943514668,21.213395603145,-15.5476309524487));
#40196=CARTESIAN_POINT('Ctrl Pts',(-20.2625820107879,21.2645425577026,-15.5518845303342));
#40197=CARTESIAN_POINT('Ctrl Pts',(-20.195201792914,21.3146979287411,-15.5560556443121));
#40198=CARTESIAN_POINT('Ctrl Pts',(-20.1253003720614,21.3615708076597,-15.5602267582901));
#40199=CARTESIAN_POINT('Ctrl Pts',(-20.0532336923063,21.4049057557434,-15.564397872268));
#40200=CARTESIAN_POINT('Ctrl Pts',(-19.9811911952218,21.4482261623666,-15.5685675865884));
#40201=CARTESIAN_POINT('Ctrl Pts',(-19.9069852761389,21.4880107590573,-15.5727373009088));
#40202=CARTESIAN_POINT('Ctrl Pts',(-19.8309999421958,21.5240480165406,-15.5769070152291));
#40203=CARTESIAN_POINT('Ctrl Pts',(-19.7550173121369,21.5600839916636,-15.5810765811732));
#40204=CARTESIAN_POINT('Ctrl Pts',(-19.6772558091333,21.5923726963449,-15.5852461471172));
#40205=CARTESIAN_POINT('Ctrl Pts',(-19.5981218233864,21.6207496704736,-15.5894157130613));
#40206=CARTESIAN_POINT('Ctrl Pts',(-19.5162055843229,21.6501243440057,-15.5937318758002));
#40207=CARTESIAN_POINT('Ctrl Pts',(-19.4328190502827,21.6753069180702,-15.5980480385391));
#40208=CARTESIAN_POINT('Ctrl Pts',(-19.3484309915969,21.6961709310559,-15.602364201278));
#40209=CARTESIAN_POINT('Ctrl Pts',(-19.2667918650467,21.7163553010131,-15.6065397654697));
#40210=CARTESIAN_POINT('Ctrl Pts',(-19.1842159325103,21.7324980994093,-15.6107153296614));
#40211=CARTESIAN_POINT('Ctrl Pts',(-19.1011369778118,21.7445371399534,-15.6148908938531));
#40212=CARTESIAN_POINT('Ctrl Pts',(-19.0138619026129,21.7571842438152,-15.6192773558656));
#40213=CARTESIAN_POINT('Ctrl Pts',(-18.9260322359072,21.7653020795901,-15.6236638178781));
#40214=CARTESIAN_POINT('Ctrl Pts',(-18.8381534037015,21.7688803858854,-15.6280502798907));
#40215=CARTESIAN_POINT('Ctrl Pts',(-18.7502745714959,21.7724586921808,-15.6324367419032));
#40216=CARTESIAN_POINT('Ctrl Pts',(-18.6623471531412,21.771497551399,-15.6368232039158));
#40217=CARTESIAN_POINT('Ctrl Pts',(-18.5748705298081,21.7660494734381,-15.6412096659283));
#40218=CARTESIAN_POINT('Ctrl Pts',(-18.491428440693,21.76085266783,-15.6453938186791));
#40219=CARTESIAN_POINT('Ctrl Pts',(-18.4080859286806,21.7515543524013,-15.6495779714299));
#40220=CARTESIAN_POINT('Ctrl Pts',(-18.3252786851367,21.7381618244142,-15.6537621241807));
#40221=CARTESIAN_POINT('Ctrl Pts',(-18.2425831161031,21.7247873576973,-15.6579406341497));
#40222=CARTESIAN_POINT('Ctrl Pts',(-18.1604218322389,21.7073297146472,-15.6621191441187));
#40223=CARTESIAN_POINT('Ctrl Pts',(-18.0792276257493,21.6858481040092,-15.6662976540877));
#40224=CARTESIAN_POINT('Ctrl Pts',(-17.9976813438716,21.6642733445281,-15.6704942829666));
#40225=CARTESIAN_POINT('Ctrl Pts',(-17.9171110155243,21.6386396626604,-15.6746909118456));
#40226=CARTESIAN_POINT('Ctrl Pts',(-17.8379469276443,21.6090594011662,-15.6788875407246));
#40227=CARTESIAN_POINT('Ctrl Pts',(-17.7592671225618,21.5796600956102,-15.6830584969125));
#40228=CARTESIAN_POINT('Ctrl Pts',(-17.6819768376045,21.546362521027,-15.6872294531003));
#40229=CARTESIAN_POINT('Ctrl Pts',(-17.6064837261605,21.509327011595,-15.6914004092882));
#40230=CARTESIAN_POINT('Ctrl Pts',(-17.5302936121915,21.4719495657518,-15.6956098745127));
#40231=CARTESIAN_POINT('Ctrl Pts',(-17.4559344801737,21.4307649580337,-15.6998193397373));
#40232=CARTESIAN_POINT('Ctrl Pts',(-17.3838034107058,21.3859871655388,-15.7040288049618));
#40233=CARTESIAN_POINT('Ctrl Pts',(-17.311672341238,21.3412093730438,-15.7082382701863));
#40234=CARTESIAN_POINT('Ctrl Pts',(-17.2417697449005,21.2928386490813,-15.7124477354108));
#40235=CARTESIAN_POINT('Ctrl Pts',(-17.1744642439897,21.2411350264762,-15.7166572006354));
#40236=CARTESIAN_POINT('',(-21.2939991231355,19.2131188547121,-15.3667098902285));
#40237=CARTESIAN_POINT('Ctrl Pts',(-21.2956374879243,19.2131202107504,-15.3667098902285));
#40238=CARTESIAN_POINT('Ctrl Pts',(-21.2969229026965,19.3573559385303,-15.3738974629702));
#40239=CARTESIAN_POINT('Ctrl Pts',(-21.2201492855026,20.3509180416766,-15.4234769712724));
#40240=CARTESIAN_POINT('Ctrl Pts',(-19.9200692925299,21.9960549863024,-15.515448415135));
#40241=CARTESIAN_POINT('Ctrl Pts',(-17.9391679704133,21.803679489263,-15.6027438707495));
#40242=CARTESIAN_POINT('Ctrl Pts',(-17.2118400551136,21.274998205827,-15.6476473908036));
#40243=CARTESIAN_POINT('Ctrl Pts',(-17.1721129955817,21.2441651167962,-15.6501589752972));
#40244=CARTESIAN_POINT('Ctrl Pts',(-17.1744642439897,21.2411350264762,-14.8500370213225));
#40245=CARTESIAN_POINT('Ctrl Pts',(-17.107823551684,21.1899421052662,-14.8542147110807));
#40246=CARTESIAN_POINT('Ctrl Pts',(-17.0437722960728,21.1355152892009,-14.8583924008388));
#40247=CARTESIAN_POINT('Ctrl Pts',(-16.9826243815685,21.0781591906325,-14.8625700905969));
#40248=CARTESIAN_POINT('Ctrl Pts',(-16.921377573247,21.0207103307072,-14.8667545368845));
#40249=CARTESIAN_POINT('Ctrl Pts',(-16.8630437949045,20.9603230647298,-14.8709389831721));
#40250=CARTESIAN_POINT('Ctrl Pts',(-16.8078981922149,20.8973368068232,-14.8751234294598));
#40251=CARTESIAN_POINT('Ctrl Pts',(-16.7883675541886,20.8750292837606,-14.8766054135491));
#40252=CARTESIAN_POINT('Ctrl Pts',(-16.7692364298418,20.8523960399785,-14.8780873976385));
#40253=CARTESIAN_POINT('Ctrl Pts',(-16.7505157350919,20.8294530178111,-14.8795693817278));
#40254=CARTESIAN_POINT('Ctrl Pts',(-16.697654666154,20.764669488533,-14.8837540161209));
#40255=CARTESIAN_POINT('Ctrl Pts',(-16.6478724513804,20.6971728954314,-14.8879386505139));
#40256=CARTESIAN_POINT('Ctrl Pts',(-16.6014597312931,20.6272881071108,-14.892123284907));
#40257=CARTESIAN_POINT('Ctrl Pts',(-16.5551130739681,20.5575027911364,-14.8963019629909));
#40258=CARTESIAN_POINT('Ctrl Pts',(-16.5121266371783,20.4853364119635,-14.9004806410748));
#40259=CARTESIAN_POINT('Ctrl Pts',(-16.4727509157821,20.4111468989768,-14.9046593191588));
#40260=CARTESIAN_POINT('Ctrl Pts',(-16.4326694128786,20.3356275922887,-14.9089128970442));
#40261=CARTESIAN_POINT('Ctrl Pts',(-16.3963296475344,20.2580122826049,-14.9131664749297));
#40262=CARTESIAN_POINT('Ctrl Pts',(-16.3639497085599,20.1787094688205,-14.9174200528151));
#40263=CARTESIAN_POINT('Ctrl Pts',(-16.3321975178868,20.1009440948281,-14.9215911667931));
#40264=CARTESIAN_POINT('Ctrl Pts',(-16.3042531677129,20.0215565094719,-14.925762280771));
#40265=CARTESIAN_POINT('Ctrl Pts',(-16.2802751807719,19.9409551434874,-14.929933394749));
#40266=CARTESIAN_POINT('Ctrl Pts',(-16.2563052398759,19.8603808240697,-14.9341031090693));
#40267=CARTESIAN_POINT('Ctrl Pts',(-16.2362991499858,19.7785939734879,-14.9382728233897));
#40268=CARTESIAN_POINT('Ctrl Pts',(-16.2203659101292,19.6960192390406,-14.9424425377101));
#40269=CARTESIAN_POINT('Ctrl Pts',(-16.2044332372457,19.6134474429568,-14.9466121036541));
#40270=CARTESIAN_POINT('Ctrl Pts',(-16.1925732125599,19.5300882706131,-14.9507816695982));
#40271=CARTESIAN_POINT('Ctrl Pts',(-16.1848436692124,19.4463762970339,-14.9549512355422));
#40272=CARTESIAN_POINT('Ctrl Pts',(-16.1768423646562,19.3597211137334,-14.9592673982811));
#40273=CARTESIAN_POINT('Ctrl Pts',(-16.1732674495782,19.2726883838098,-14.9635835610201));
#40274=CARTESIAN_POINT('Ctrl Pts',(-16.1741243927921,19.185763605208,-14.967899723759));
#40275=CARTESIAN_POINT('Ctrl Pts',(-16.174953421171,19.1016703921264,-14.9720752879507));
#40276=CARTESIAN_POINT('Ctrl Pts',(-16.1799299313355,19.0176786727672,-14.9762508521424));
#40277=CARTESIAN_POINT('Ctrl Pts',(-16.1890058822548,18.9342240244489,-14.980426416334));
#40278=CARTESIAN_POINT('Ctrl Pts',(-16.198540237879,18.8465542802385,-14.9848128783466));
#40279=CARTESIAN_POINT('Ctrl Pts',(-16.2125989501167,18.7594778642492,-14.9891993403591));
#40280=CARTESIAN_POINT('Ctrl Pts',(-16.2310658163554,18.6734867700759,-14.9935858023717));
#40281=CARTESIAN_POINT('Ctrl Pts',(-16.2495326825942,18.5874956759026,-14.9979722643842));
#40282=CARTESIAN_POINT('Ctrl Pts',(-16.2724074784504,18.5025904439986,-15.0023587263968));
#40283=CARTESIAN_POINT('Ctrl Pts',(-16.2995147249237,18.4192415485537,-15.0067451884093));
#40284=CARTESIAN_POINT('Ctrl Pts',(-16.3253747268042,18.3397276593411,-15.0109298228024));
#40285=CARTESIAN_POINT('Ctrl Pts',(-16.3551825113727,18.2613340692511,-15.0151144571954));
#40286=CARTESIAN_POINT('Ctrl Pts',(-16.3888222337464,18.1844810061817,-15.0192990915885));
#40287=CARTESIAN_POINT('Ctrl Pts',(-16.4224140741391,18.1077373339352,-15.0234777696724));
#40288=CARTESIAN_POINT('Ctrl Pts',(-16.4598268355143,18.0325302510435,-15.0276564477563));
#40289=CARTESIAN_POINT('Ctrl Pts',(-16.5008951440191,17.9592641244279,-15.0318351258403));
#40290=CARTESIAN_POINT('Ctrl Pts',(-16.5426995724385,17.8846847551482,-15.0360887037257));
#40291=CARTESIAN_POINT('Ctrl Pts',(-16.5882917392508,17.8121170683453,-15.0403422816112));
#40292=CARTESIAN_POINT('Ctrl Pts',(-16.6374462088683,17.7419655548996,-15.0445958594966));
#40293=CARTESIAN_POINT('Ctrl Pts',(-16.6856477231752,17.6731740654315,-15.0487669734745));
#40294=CARTESIAN_POINT('Ctrl Pts',(-16.7372743723595,17.606706294976,-15.0529380874525));
#40295=CARTESIAN_POINT('Ctrl Pts',(-16.792068536157,17.5429166118756,-15.0571092014304));
#40296=CARTESIAN_POINT('Ctrl Pts',(-16.8468443132437,17.4791483340195,-15.0612789157508));
#40297=CARTESIAN_POINT('Ctrl Pts',(-16.9047851945213,17.4180567074448,-15.0654486300712));
#40298=CARTESIAN_POINT('Ctrl Pts',(-16.9655931179199,17.3599632366126,-15.0696183443915));
#40299=CARTESIAN_POINT('Ctrl Pts',(-17.0263988775115,17.3018718329955,-15.0737879103356));
#40300=CARTESIAN_POINT('Ctrl Pts',(-17.0900711431583,17.2467786901665,-15.0779574762796));
#40301=CARTESIAN_POINT('Ctrl Pts',(-17.1562758100197,17.1949676638628,-15.0821270422237));
#40302=CARTESIAN_POINT('Ctrl Pts',(-17.2248081512957,17.14133502579,-15.0864432049626));
#40303=CARTESIAN_POINT('Ctrl Pts',(-17.2960538702051,17.0912199219507,-15.0907593677015));
#40304=CARTESIAN_POINT('Ctrl Pts',(-17.3696076999732,17.0448897415811,-15.0950755304404));
#40305=CARTESIAN_POINT('Ctrl Pts',(-17.440765521473,17.000068761964,-15.0992510946321));
#40306=CARTESIAN_POINT('Ctrl Pts',(-17.5140829560414,16.9587900948024,-15.1034266588238));
#40307=CARTESIAN_POINT('Ctrl Pts',(-17.5891677483861,16.9212491149331,-15.1076022230154));
#40308=CARTESIAN_POINT('Ctrl Pts',(-17.6680448950951,16.8818120294158,-15.111988685028));
#40309=CARTESIAN_POINT('Ctrl Pts',(-17.74887209509,16.8465003691281,-15.1163751470405));
#40310=CARTESIAN_POINT('Ctrl Pts',(-17.831172761347,16.8154827328641,-15.120761609053));
#40311=CARTESIAN_POINT('Ctrl Pts',(-17.913473427604,16.7844650966001,-15.1251480710656));
#40312=CARTESIAN_POINT('Ctrl Pts',(-17.9972469842329,16.7577415882257,-15.1295345330781));
#40313=CARTESIAN_POINT('Ctrl Pts',(-18.0820028534396,16.7354193164275,-15.1339209950906));
#40314=CARTESIAN_POINT('Ctrl Pts',(-18.1628589794658,16.7141241254443,-15.1381056294837));
#40315=CARTESIAN_POINT('Ctrl Pts',(-18.2449099711144,16.6967547916185,-15.1422902638767));
#40316=CARTESIAN_POINT('Ctrl Pts',(-18.3277397785879,16.6834413691275,-15.1464748982698));
#40317=CARTESIAN_POINT('Ctrl Pts',(-18.4104516880828,16.6701468966455,-15.1506535763537));
#40318=CARTESIAN_POINT('Ctrl Pts',(-18.4939397611591,16.66089694071,-15.1548322544377));
#40319=CARTESIAN_POINT('Ctrl Pts',(-18.5777744754985,16.6557713242267,-15.1590109325216));
#40320=CARTESIAN_POINT('Ctrl Pts',(-18.6631118668416,16.6505538347517,-15.163264510407));
#40321=CARTESIAN_POINT('Ctrl Pts',(-18.7488079825292,16.6496101194126,-15.1675180882925));
#40322=CARTESIAN_POINT('Ctrl Pts',(-18.8344006857351,16.652969565798,-15.1717716661779));
#40323=CARTESIAN_POINT('Ctrl Pts',(-18.9183340073688,16.6562638827597,-15.1759427801559));
#40324=CARTESIAN_POINT('Ctrl Pts',(-19.0021674095958,16.6636959811426,-15.1801138941338));
#40325=CARTESIAN_POINT('Ctrl Pts',(-19.085463479757,16.6752410559367,-15.1842850081118));
#40326=CARTESIAN_POINT('Ctrl Pts',(-19.1687315991175,16.6867822566694,-15.1884547224321));
#40327=CARTESIAN_POINT('Ctrl Pts',(-19.2514622892072,16.70243362971,-15.1926244367525));
#40328=CARTESIAN_POINT('Ctrl Pts',(-19.3332238803081,16.7221185762941,-15.1967941510729));
#40329=CARTESIAN_POINT('Ctrl Pts',(-19.4149825619807,16.7418028224032,-15.2009637170169));
#40330=CARTESIAN_POINT('Ctrl Pts',(-19.4957717661756,16.7655202481684,-15.205133282961));
#40331=CARTESIAN_POINT('Ctrl Pts',(-19.5751719705257,16.7931435700187,-15.209302848905));
#40332=CARTESIAN_POINT('Ctrl Pts',(-19.6573637881101,16.8217380937883,-15.2136190116439));
#40333=CARTESIAN_POINT('Ctrl Pts',(-19.7380666159157,16.8545181133117,-15.2179351743828));
#40334=CARTESIAN_POINT('Ctrl Pts',(-19.8168362586914,16.891287596088,-15.2222513371218));
#40335=CARTESIAN_POINT('Ctrl Pts',(-19.8930399886387,16.9268593168303,-15.2264269013134));
#40336=CARTESIAN_POINT('Ctrl Pts',(-19.9674341519876,16.966164316944,-15.2306024655051));
#40337=CARTESIAN_POINT('Ctrl Pts',(-20.0396421490694,17.0089785244977,-15.2347780296968));
#40338=CARTESIAN_POINT('Ctrl Pts',(-20.1154972004257,17.0539551758939,-15.2391644917093));
#40339=CARTESIAN_POINT('Ctrl Pts',(-20.1889389488847,17.1028045279329,-15.2435509537219));
#40340=CARTESIAN_POINT('Ctrl Pts',(-20.2595676620248,17.1552171056787,-15.2479374157344));
#40341=CARTESIAN_POINT('Ctrl Pts',(-20.330196375165,17.2076296834245,-15.252323877747));
#40342=CARTESIAN_POINT('Ctrl Pts',(-20.3980116539332,17.2636050588652,-15.2567103397595));
#40343=CARTESIAN_POINT('Ctrl Pts',(-20.4626578964189,17.3227887096121,-15.2610968017721));
#40344=CARTESIAN_POINT('Ctrl Pts',(-20.5234100187947,17.3784072924496,-15.2652190348167));
#40345=CARTESIAN_POINT('Ctrl Pts',(-20.5816044022757,17.4370795204071,-15.2693412678613));
#40346=CARTESIAN_POINT('Ctrl Pts',(-20.6369112461388,17.498537215202,-15.2734635009059));
#40347=CARTESIAN_POINT('Ctrl Pts',(-20.6921256485485,17.5598921878337,-15.2775788439313));
#40348=CARTESIAN_POINT('Ctrl Pts',(-20.7444617859859,17.6240230272318,-15.2816941869567));
#40349=CARTESIAN_POINT('Ctrl Pts',(-20.793624524071,17.6906228034315,-15.2858095299821));
#40350=CARTESIAN_POINT('Ctrl Pts',(-20.8427410076366,17.7571599195604,-15.2899210011074));
#40351=CARTESIAN_POINT('Ctrl Pts',(-20.8886897335868,17.8261609852054,-15.2940324722326));
#40352=CARTESIAN_POINT('Ctrl Pts',(-20.9312146121396,17.8972846776412,-15.2981439433579));
#40353=CARTESIAN_POINT('Ctrl Pts',(-20.9737131282073,17.9683642783043,-15.3022528656552));
#40354=CARTESIAN_POINT('Ctrl Pts',(-21.0127917657825,18.0415634879279,-15.3063617879526));
#40355=CARTESIAN_POINT('Ctrl Pts',(-21.0482376124066,18.1165118669796,-15.3104707102499));
#40356=CARTESIAN_POINT('Ctrl Pts',(-21.0836728562224,18.1914378269505,-15.3145784034579));
#40357=CARTESIAN_POINT('Ctrl Pts',(-21.1154772648512,18.2681114878987,-15.3186860966658));
#40358=CARTESIAN_POINT('Ctrl Pts',(-21.1434845038954,18.3461390715913,-15.3227937898737));
#40359=CARTESIAN_POINT('Ctrl Pts',(-21.1715053065244,18.4242044431482,-15.3269034723903));
#40360=CARTESIAN_POINT('Ctrl Pts',(-21.1957251016689,18.5036246009545,-15.331013154907));
#40361=CARTESIAN_POINT('Ctrl Pts',(-21.2160265895475,18.5839880313906,-15.3351228374236));
#40362=CARTESIAN_POINT('Ctrl Pts',(-21.2363332616047,18.6643719833958,-15.339233569387));
#40363=CARTESIAN_POINT('Ctrl Pts',(-21.2527195357628,18.7456992225568,-15.3433443013503));
#40364=CARTESIAN_POINT('Ctrl Pts',(-21.2651191757883,18.827547632741,-15.3474550333136));
#40365=CARTESIAN_POINT('Ctrl Pts',(-21.2775338661873,18.9094953884813,-15.3515707547807));
#40366=CARTESIAN_POINT('Ctrl Pts',(-21.2859522113273,18.9919651056503,-15.3556864762478));
#40367=CARTESIAN_POINT('Ctrl Pts',(-21.2903598951031,19.0745299054426,-15.3598021977149));
#40368=CARTESIAN_POINT('Ctrl Pts',(-21.292825799276,19.1207212600627,-15.3621047618861));
#40369=CARTESIAN_POINT('Ctrl Pts',(-21.294037342402,19.1669423575626,-15.3644073260573));
#40370=CARTESIAN_POINT('Ctrl Pts',(-21.2939991231355,19.2131188547121,-15.3667098902285));
#40371=CARTESIAN_POINT('Origin',(-18.734,19.211,1.76670989022852));
#40372=CARTESIAN_POINT('',(-17.1770151058749,21.2378231662188,-14.0501277782861));
#40373=CARTESIAN_POINT('',(-17.1718944362858,21.2444720185936,-14.1167030376167));
#40374=CARTESIAN_POINT('',(-17.1744642439897,21.2411350264762,1.76670989022852));
#40375=CARTESIAN_POINT('',(-21.2941234937244,19.2098698166564,-14.6332901097715));
#40376=CARTESIAN_POINT('Ctrl Pts',(-17.1718944362858,21.2444720185936,-14.1167030376167));
#40377=CARTESIAN_POINT('Ctrl Pts',(-16.5081485897239,20.7333156289599,-14.1585606225553));
#40378=CARTESIAN_POINT('Ctrl Pts',(-15.721016264389,18.9872885886645,-14.2428101430544));
#40379=CARTESIAN_POINT('Ctrl Pts',(-17.2790524810781,16.55649072778,-14.3694515991139));
#40380=CARTESIAN_POINT('Ctrl Pts',(-20.1784867160069,16.5507838647211,-14.4966274057954));
#40381=CARTESIAN_POINT('Ctrl Pts',(-21.2671018326456,18.2345793421635,-14.5845735760146));
#40382=CARTESIAN_POINT('Ctrl Pts',(-21.2979709281649,19.1465375840163,-14.6301278106733));
#40383=CARTESIAN_POINT('Ctrl Pts',(-21.2976211493107,19.2098682725933,-14.6332901097715));
#40384=CARTESIAN_POINT('Ctrl Pts',(-21.2939997505486,19.2098698712836,-14.6332901097715));
#40385=CARTESIAN_POINT('Ctrl Pts',(-21.2940362985033,19.2926593390013,-14.6374299052976));
#40386=CARTESIAN_POINT('Ctrl Pts',(-21.2900525381051,19.3756125071059,-14.6415697008237));
#40387=CARTESIAN_POINT('Ctrl Pts',(-21.2820270867845,19.4583013647603,-14.6457094963498));
#40388=CARTESIAN_POINT('Ctrl Pts',(-21.2740124509524,19.5408787868902,-14.6498437128862));
#40389=CARTESIAN_POINT('Ctrl Pts',(-21.2619669829652,19.623192141297,-14.6539779294226));
#40390=CARTESIAN_POINT('Ctrl Pts',(-21.2459213201026,19.7048130026779,-14.658112145959));
#40391=CARTESIAN_POINT('Ctrl Pts',(-21.2298921267197,19.7863500873319,-14.6622421190811));
#40392=CARTESIAN_POINT('Ctrl Pts',(-21.209870984755,19.8671956313595,-14.6663720922032));
#40393=CARTESIAN_POINT('Ctrl Pts',(-21.1859402178855,19.9469274202771,-14.6705020653253));
#40394=CARTESIAN_POINT('Ctrl Pts',(-21.1620224032908,20.026616055206,-14.6746298031431));
#40395=CARTESIAN_POINT('Ctrl Pts',(-21.1341992976676,20.105191681447,-14.6787575409609));
#40396=CARTESIAN_POINT('Ctrl Pts',(-21.1026037847566,20.1822446194635,-14.6828852787786));
#40397=CARTESIAN_POINT('Ctrl Pts',(-21.0710154147152,20.2592801379466,-14.6870120834293));
#40398=CARTESIAN_POINT('Ctrl Pts',(-21.0356565094082,20.3347932165768,-14.69113888808));
#40399=CARTESIAN_POINT('Ctrl Pts',(-20.9967085276621,20.4083930511094,-14.6952656927306));
#40400=CARTESIAN_POINT('Ctrl Pts',(-20.9577570758468,20.481999443017,-14.6993928650588));
#40401=CARTESIAN_POINT('Ctrl Pts',(-20.915216134864,20.5536918375766,-14.703520037387));
#40402=CARTESIAN_POINT('Ctrl Pts',(-20.8693129406042,20.6231043324372,-14.7076472097152));
#40403=CARTESIAN_POINT('Ctrl Pts',(-20.82336222789,20.6925886823078,-14.7117786544443));
#40404=CARTESIAN_POINT('Ctrl Pts',(-20.7740425759679,20.7597880294049,-14.7159100991735));
#40405=CARTESIAN_POINT('Ctrl Pts',(-20.7216239583874,20.8243663564251,-14.7200415439026));
#40406=CARTESIAN_POINT('Ctrl Pts',(-20.6691749218121,20.8889821588287,-14.7241753861462));
#40407=CARTESIAN_POINT('Ctrl Pts',(-20.6136236562298,20.9509735655346,-14.7283092283899));
#40408=CARTESIAN_POINT('Ctrl Pts',(-20.5552780488243,21.0100403744415,-14.7324430706335));
#40409=CARTESIAN_POINT('Ctrl Pts',(-20.496836459412,21.0692043517748,-14.7365837132944));
#40410=CARTESIAN_POINT('Ctrl Pts',(-20.4355917013479,21.1254338132407,-14.7407243559553));
#40411=CARTESIAN_POINT('Ctrl Pts',(-20.3718854170609,21.1784682616447,-14.7448649986162));
#40412=CARTESIAN_POINT('Ctrl Pts',(-20.340529452726,21.2045715933849,-14.7469030054635));
#40413=CARTESIAN_POINT('Ctrl Pts',(-20.3085776248467,21.2299015689541,-14.7489410123109));
#40414=CARTESIAN_POINT('Ctrl Pts',(-20.2760730898184,21.2544310817001,-14.7509790191583));
#40415=CARTESIAN_POINT('Ctrl Pts',(-20.2093316088543,21.3047974692387,-14.7551636535513));
#40416=CARTESIAN_POINT('Ctrl Pts',(-20.1399957689001,21.3519843348468,-14.7593482879444));
#40417=CARTESIAN_POINT('Ctrl Pts',(-20.0684012262927,21.3957135664129,-14.7635329223374));
#40418=CARTESIAN_POINT('Ctrl Pts',(-19.9969085896549,21.4393805548305,-14.7677116004214));
#40419=CARTESIAN_POINT('Ctrl Pts',(-19.9231640255691,21.4795994471402,-14.7718902785053));
#40420=CARTESIAN_POINT('Ctrl Pts',(-19.8475347050064,21.5161335017188,-14.7760689565893));
#40421=CARTESIAN_POINT('Ctrl Pts',(-19.7705497832267,21.553322402969,-14.7803225344747));
#40422=CARTESIAN_POINT('Ctrl Pts',(-19.6916122567004,21.5866927752846,-14.7845761123602));
#40423=CARTESIAN_POINT('Ctrl Pts',(-19.6111386006649,21.6160421774313,-14.7888296902456));
#40424=CARTESIAN_POINT('Ctrl Pts',(-19.532225083483,21.6448225841468,-14.7930008042235));
#40425=CARTESIAN_POINT('Ctrl Pts',(-19.4518349191,21.6697363732163,-14.7971719182015));
#40426=CARTESIAN_POINT('Ctrl Pts',(-19.3703822558334,21.6906406240543,-14.8013430321794));
#40427=CARTESIAN_POINT('Ctrl Pts',(-19.2889569247947,21.711537860269,-14.8055127464998));
#40428=CARTESIAN_POINT('Ctrl Pts',(-19.2064702481715,21.728428116053,-14.8096824608202));
#40429=CARTESIAN_POINT('Ctrl Pts',(-19.1233507011891,21.7412185738555,-14.8138521751405));
#40430=CARTESIAN_POINT('Ctrl Pts',(-19.0402341119568,21.7540085765187,-14.8180217410846));
#40431=CARTESIAN_POINT('Ctrl Pts',(-18.9564851519519,21.7626990021399,-14.8221913070286));
#40432=CARTESIAN_POINT('Ctrl Pts',(-18.8725402767196,21.7672485387236,-14.8263608729727));
#40433=CARTESIAN_POINT('Ctrl Pts',(-18.7856440032314,21.7719580314011,-14.8306770357116));
#40434=CARTESIAN_POINT('Ctrl Pts',(-18.6985383080786,21.7722300013651,-14.8349931984505));
#40435=CARTESIAN_POINT('Ctrl Pts',(-18.6117085473887,21.7680773943348,-14.8393093611894));
#40436=CARTESIAN_POINT('Ctrl Pts',(-18.5277072570202,21.7640600580418,-14.8434849253811));
#40437=CARTESIAN_POINT('Ctrl Pts',(-18.4439646643002,21.7559020718402,-14.8476604895728));
#40438=CARTESIAN_POINT('Ctrl Pts',(-18.3609142114856,21.7436679597627,-14.8518360537645));
#40439=CARTESIAN_POINT('Ctrl Pts',(-18.2736690777334,21.7308159317681,-14.856222515777));
#40440=CARTESIAN_POINT('Ctrl Pts',(-18.187188413865,21.713465300997,-14.8606089777895));
#40441=CARTESIAN_POINT('Ctrl Pts',(-18.1019594530762,21.6917508434029,-14.8649954398021));
#40442=CARTESIAN_POINT('Ctrl Pts',(-18.0167304922875,21.6700363858088,-14.8693819018146));
#40443=CARTESIAN_POINT('Ctrl Pts',(-17.932753766134,21.6439583461084,-14.8737683638271));
#40444=CARTESIAN_POINT('Ctrl Pts',(-17.8504927560607,21.613709917969,-14.8781548258396));
#40445=CARTESIAN_POINT('Ctrl Pts',(-17.7720269461522,21.5848570335916,-14.8823389137099));
#40446=CARTESIAN_POINT('Ctrl Pts',(-17.6948300019125,21.5521027093235,-14.8865230015802));
#40447=CARTESIAN_POINT('Ctrl Pts',(-17.6193172941086,21.5155785873314,-14.8907070894505));
#40448=CARTESIAN_POINT('Ctrl Pts',(-17.5409562028295,21.4776767541096,-14.8950490035609));
#40449=CARTESIAN_POINT('Ctrl Pts',(-17.4644094236413,21.4357151583199,-14.8993909176712));
#40450=CARTESIAN_POINT('Ctrl Pts',(-17.3901227910456,21.3898974384429,-14.9037328317816));
#40451=CARTESIAN_POINT('Ctrl Pts',(-17.31583615845,21.3440797185659,-14.9080747458919));
#40452=CARTESIAN_POINT('Ctrl Pts',(-17.2438101840022,21.2944061003571,-14.9124166600022));
#40453=CARTESIAN_POINT('Ctrl Pts',(-17.1744642439897,21.2411350264762,-14.9167585741126));
#40454=CARTESIAN_POINT('',(-21.2936354898062,19.2115601738724,-14.5667099150531));
#40455=CARTESIAN_POINT('Ctrl Pts',(-21.2939999386838,19.2115603024813,-14.5667099174733));
#40456=CARTESIAN_POINT('Ctrl Pts',(-21.2939802627011,19.301459091566,-14.5711571992722));
#40457=CARTESIAN_POINT('Ctrl Pts',(-21.2892209204019,19.3912344818061,-14.5756044810712));
#40458=CARTESIAN_POINT('Ctrl Pts',(-21.2797861099485,19.4803939167712,-14.5800517628701));
#40459=CARTESIAN_POINT('Ctrl Pts',(-21.270316767046,19.5698796851229,-14.584515322212));
#40460=CARTESIAN_POINT('Ctrl Pts',(-21.2561377674645,19.6587446305213,-14.5889788815539));
#40461=CARTESIAN_POINT('Ctrl Pts',(-21.2373647797492,19.7465042292186,-14.5934424408958));
#40462=CARTESIAN_POINT('Ctrl Pts',(-21.2185553401057,19.8344342326829,-14.5979146672303));
#40463=CARTESIAN_POINT('Ctrl Pts',(-21.1951342035234,19.9212542602487,-14.6023868935647));
#40464=CARTESIAN_POINT('Ctrl Pts',(-21.1672666877215,20.0064955854214,-14.6068591198992));
#40465=CARTESIAN_POINT('Ctrl Pts',(-21.1393161596827,20.0919908289243,-14.6113446681786));
#40466=CARTESIAN_POINT('Ctrl Pts',(-21.1068928974848,20.1758976314735,-14.615830216458));
#40467=CARTESIAN_POINT('Ctrl Pts',(-21.0702104967872,20.2577666954491,-14.6203157647375));
#40468=CARTESIAN_POINT('Ctrl Pts',(-21.0568477853949,20.2875900617789,-14.6219497659466));
#40469=CARTESIAN_POINT('Ctrl Pts',(-21.0429203172376,20.3171432681498,-14.6235837671558));
#40470=CARTESIAN_POINT('Ctrl Pts',(-21.0284398795323,20.3464054955,-14.6252177683649));
#40471=CARTESIAN_POINT('Ctrl Pts',(-20.9913558570061,20.4213452949944,-14.6294024027579));
#40472=CARTESIAN_POINT('Ctrl Pts',(-20.9505274948145,20.4946058152548,-14.633587037151));
#40473=CARTESIAN_POINT('Ctrl Pts',(-20.9061301751472,20.5657879916116,-14.637771671544));
#40474=CARTESIAN_POINT('Ctrl Pts',(-20.8617960495691,20.636868848951,-14.641950349628));
#40475=CARTESIAN_POINT('Ctrl Pts',(-20.8139032983065,20.7058768514385,-14.6461290277119));
#40476=CARTESIAN_POINT('Ctrl Pts',(-20.7626740190628,20.7724357893874,-14.6503077057959));
#40477=CARTESIAN_POINT('Ctrl Pts',(-20.7105264918065,20.8401877484639,-14.6545612836813));
#40478=CARTESIAN_POINT('Ctrl Pts',(-20.6549218593555,20.9054015483268,-14.6588148615668));
#40479=CARTESIAN_POINT('Ctrl Pts',(-20.5961416680528,20.9677095400496,-14.6630684394522));
#40480=CARTESIAN_POINT('Ctrl Pts',(-20.5385010454587,21.0288095697688,-14.6672395534301));
#40481=CARTESIAN_POINT('Ctrl Pts',(-20.4778072242622,21.0871151053885,-14.6714106674081));
#40482=CARTESIAN_POINT('Ctrl Pts',(-20.4143663508875,21.1423127470208,-14.6755817813861));
#40483=CARTESIAN_POINT('Ctrl Pts',(-20.3509467657105,21.1974918665513,-14.6797514957064));
#40484=CARTESIAN_POINT('Ctrl Pts',(-20.2847823058331,21.2495648615672,-14.6839212100268));
#40485=CARTESIAN_POINT('Ctrl Pts',(-20.2162143833073,21.2982566976577,-14.6880909243472));
#40486=CARTESIAN_POINT('Ctrl Pts',(-20.1476489007224,21.3469468010838,-14.6922604902912));
#40487=CARTESIAN_POINT('Ctrl Pts',(-20.0766805011099,21.3922557191444,-14.6964300562353));
#40488=CARTESIAN_POINT('Ctrl Pts',(-20.0036808175629,21.433950881489,-14.7005996221793));
#40489=CARTESIAN_POINT('Ctrl Pts',(-19.9281145551974,21.477111994305,-14.7049157849182));
#40490=CARTESIAN_POINT('Ctrl Pts',(-19.850371969323,21.5164002423867,-14.7092319476572));
#40491=CARTESIAN_POINT('Ctrl Pts',(-19.7708927266886,21.5516096371117,-14.7135481103961));
#40492=CARTESIAN_POINT('Ctrl Pts',(-19.6940025120233,21.5856720895069,-14.7177236745878));
#40493=CARTESIAN_POINT('Ctrl Pts',(-19.6154875027973,21.6159172197028,-14.7218992387794));
#40494=CARTESIAN_POINT('Ctrl Pts',(-19.5357640795052,21.6422084157503,-14.7260748029711));
#40495=CARTESIAN_POINT('Ctrl Pts',(-19.4520140156271,21.6698275176088,-14.7304612649837));
#40496=CARTESIAN_POINT('Ctrl Pts',(-19.3669308187544,21.6930826078309,-14.7348477269962));
#40497=CARTESIAN_POINT('Ctrl Pts',(-19.2810104439706,21.7118757614458,-14.7392341890088));
#40498=CARTESIAN_POINT('Ctrl Pts',(-19.1950900691869,21.7306689150607,-14.7436206510213));
#40499=CARTESIAN_POINT('Ctrl Pts',(-19.1083331013483,21.7450001125529,-14.7480071130338));
#40500=CARTESIAN_POINT('Ctrl Pts',(-19.021240449396,21.7548342957494,-14.7523935750464));
#40501=CARTESIAN_POINT('Ctrl Pts',(-18.9381783893849,21.7642133592698,-14.756577034417));
#40502=CARTESIAN_POINT('Ctrl Pts',(-18.8545019430903,21.7695373443223,-14.7607604937876));
#40503=CARTESIAN_POINT('Ctrl Pts',(-18.7706412277764,21.7707377639959,-14.7649439531582));
#40504=CARTESIAN_POINT('Ctrl Pts',(-18.6868897531641,21.7719366199495,-14.7691219629684));
#40505=CARTESIAN_POINT('Ctrl Pts',(-18.6029549415235,21.7690225671098,-14.7732999727786));
#40506=CARTESIAN_POINT('Ctrl Pts',(-18.5192731319562,21.7619787086803,-14.7774779825888));
#40507=CARTESIAN_POINT('Ctrl Pts',(-18.4356752189388,21.7549419121848,-14.7816518036677));
#40508=CARTESIAN_POINT('Ctrl Pts',(-18.3523302600542,21.7437835702215,-14.7858256247467));
#40509=CARTESIAN_POINT('Ctrl Pts',(-18.2696743384136,21.7285388139992,-14.7899994458256));
#40510=CARTESIAN_POINT('Ctrl Pts',(-18.1870764857601,21.7133047678086,-14.7941703346336));
#40511=CARTESIAN_POINT('Ctrl Pts',(-18.1051671597161,21.6939900938571,-14.7983412234415));
#40512=CARTESIAN_POINT('Ctrl Pts',(-18.0243757041524,21.6706815563692,-14.8025121122494));
#40513=CARTESIAN_POINT('Ctrl Pts',(-17.9435959999342,21.6473764091739,-14.8066823943898));
#40514=CARTESIAN_POINT('Ctrl Pts',(-17.8639342884426,21.6200786673611,-14.8108526765302));
#40515=CARTESIAN_POINT('Ctrl Pts',(-17.7858071130466,21.5889256189231,-14.8150229586706));
#40516=CARTESIAN_POINT('Ctrl Pts',(-17.7076898406079,21.5577765192687,-14.8191927122097));
#40517=CARTESIAN_POINT('Ctrl Pts',(-17.6311071429207,21.5227732602774,-14.8233624657488));
#40518=CARTESIAN_POINT('Ctrl Pts',(-17.556456222726,21.4841015491181,-14.8275322192879));
#40519=CARTESIAN_POINT('Ctrl Pts',(-17.4817531860181,21.4454028398357,-14.831704883883));
#40520=CARTESIAN_POINT('Ctrl Pts',(-17.408985028084,21.403030778009,-14.8358775484782));
#40521=CARTESIAN_POINT('Ctrl Pts',(-17.3385243274801,21.3572170550541,-14.8400502130733));
#40522=CARTESIAN_POINT('Ctrl Pts',(-17.2823110461754,21.3206670395985,-14.8433791491564));
#40523=CARTESIAN_POINT('Ctrl Pts',(-17.2275659863547,21.2819274195164,-14.8467080852395));
#40524=CARTESIAN_POINT('Ctrl Pts',(-17.1744642439897,21.2411350264762,-14.8500370213225));
#40525=CARTESIAN_POINT('Ctrl Pts',(-17.1770151058749,21.2378231662188,-14.0501277782861));
#40526=CARTESIAN_POINT('Ctrl Pts',(-16.8231471434315,20.9653100508297,-14.0722566994038));
#40527=CARTESIAN_POINT('Ctrl Pts',(-15.9876140958797,19.9142911360265,-14.136777556082));
#40528=CARTESIAN_POINT('Ctrl Pts',(-16.2435265724331,17.4902926599815,-14.2436903483207));
#40529=CARTESIAN_POINT('Ctrl Pts',(-18.8327965343378,16.1855197260249,-14.3708661550021));
#40530=CARTESIAN_POINT('Ctrl Pts',(-20.9482576099774,17.4308694729993,-14.4785393356381));
#40531=CARTESIAN_POINT('Ctrl Pts',(-21.2889976010488,18.7496082874005,-14.5438205807135));
#40532=CARTESIAN_POINT('Ctrl Pts',(-21.2898971100035,19.211558854651,-14.5667098902285));
#40533=CARTESIAN_POINT('Origin',(-18.734,19.211,1.76670989022852));
#40534=CARTESIAN_POINT('',(-17.1744642439897,21.2411350264762,-13.2501880045741));
#40535=CARTESIAN_POINT('',(-17.1744642439897,21.2411350264762,-13.3166223692584));
#40536=CARTESIAN_POINT('',(-17.1744642439897,21.2411350264762,1.76670989022852));
#40537=CARTESIAN_POINT('',(-21.2939989424941,19.2133268925441,-13.8332901097715));
#40538=CARTESIAN_POINT('Ctrl Pts',(-17.1744642439897,21.2411350264762,-13.3166223692584));
#40539=CARTESIAN_POINT('Ctrl Pts',(-17.1077897971069,21.1899161752323,-13.3207986424165));
#40540=CARTESIAN_POINT('Ctrl Pts',(-17.0436959027707,21.1354513017812,-13.3249749155745));
#40541=CARTESIAN_POINT('Ctrl Pts',(-16.9824997973296,21.0780423241173,-13.3291511887325));
#40542=CARTESIAN_POINT('Ctrl Pts',(-16.9211960076474,21.0205323262636,-13.3333348107047));
#40543=CARTESIAN_POINT('Ctrl Pts',(-16.8628005132386,20.960068206441,-13.3375184326769));
#40544=CARTESIAN_POINT('Ctrl Pts',(-16.8075924183714,20.8969874938575,-13.3417020546491));
#40545=CARTESIAN_POINT('Ctrl Pts',(-16.7620957686836,20.8450030685775,-13.3451497516536));
#40546=CARTESIAN_POINT('Ctrl Pts',(-16.7187631096113,20.7912423596748,-13.348597448658));
#40547=CARTESIAN_POINT('Ctrl Pts',(-16.6777284049171,20.7359088914604,-13.3520451456625));
#40548=CARTESIAN_POINT('Ctrl Pts',(-16.6279226254793,20.6687480203406,-13.3562297800555));
#40549=CARTESIAN_POINT('Ctrl Pts',(-16.5813179797009,20.5990195040796,-13.3604144144486));
#40550=CARTESIAN_POINT('Ctrl Pts',(-16.5381897594128,20.5270613159471,-13.3645990488416));
#40551=CARTESIAN_POINT('Ctrl Pts',(-16.4951229268081,20.4552055513886,-13.3687777269256));
#40552=CARTESIAN_POINT('Ctrl Pts',(-16.4555229253634,20.3811268100629,-13.3729564050095));
#40553=CARTESIAN_POINT('Ctrl Pts',(-16.4196234139921,20.3051942323638,-13.3771350830935));
#40554=CARTESIAN_POINT('Ctrl Pts',(-16.38308042968,20.2279006177814,-13.3813886609789));
#40555=CARTESIAN_POINT('Ctrl Pts',(-16.350372190068,20.1486864403631,-13.3856422388643));
#40556=CARTESIAN_POINT('Ctrl Pts',(-16.3216976420462,20.0679698558353,-13.3898958167498));
#40557=CARTESIAN_POINT('Ctrl Pts',(-16.2935790060915,19.9888181198039,-13.3940669307277));
#40558=CARTESIAN_POINT('Ctrl Pts',(-16.2693392165556,19.9082221644551,-13.3982380447057));
#40559=CARTESIAN_POINT('Ctrl Pts',(-16.2491177212504,19.8265973202963,-13.4024091586836));
#40560=CARTESIAN_POINT('Ctrl Pts',(-16.2289030114632,19.7449998661423,-13.406578873004));
#40561=CARTESIAN_POINT('Ctrl Pts',(-16.2127040285387,19.6623746550199,-13.4107485873244));
#40562=CARTESIAN_POINT('Ctrl Pts',(-16.2006099990479,19.5791509243174,-13.4149183016448));
#40563=CARTESIAN_POINT('Ctrl Pts',(-16.1885163999145,19.4959301550723,-13.4190878675888));
#40564=CARTESIAN_POINT('Ctrl Pts',(-16.1805275290999,19.4121113639662,-13.4232574335329));
#40565=CARTESIAN_POINT('Ctrl Pts',(-16.1766810426043,19.3281313371591,-13.4274269994769));
#40566=CARTESIAN_POINT('Ctrl Pts',(-16.1726993183887,19.24119867621,-13.4317431622158));
#40567=CARTESIAN_POINT('Ctrl Pts',(-16.1731567148618,19.154093757381,-13.4360593249547));
#40568=CARTESIAN_POINT('Ctrl Pts',(-16.1780362227548,19.0673018113875,-13.4403754876937));
#40569=CARTESIAN_POINT('Ctrl Pts',(-16.1827567811915,18.9833371039057,-13.4445510518853));
#40570=CARTESIAN_POINT('Ctrl Pts',(-16.1916156782438,18.8996657556595,-13.448726616077));
#40571=CARTESIAN_POINT('Ctrl Pts',(-16.2045447628248,18.8167206534358,-13.4529021802687));
#40572=CARTESIAN_POINT('Ctrl Pts',(-16.2181268647321,18.729586191282,-13.4572886422812));
#40573=CARTESIAN_POINT('Ctrl Pts',(-16.236201010622,18.643253840094,-13.4616751042938));
#40574=CARTESIAN_POINT('Ctrl Pts',(-16.2586283495454,18.5582096874756,-13.4660615663063));
#40575=CARTESIAN_POINT('Ctrl Pts',(-16.2810556884688,18.4731655348573,-13.4704480283188));
#40576=CARTESIAN_POINT('Ctrl Pts',(-16.3078359712666,18.3894101102965,-13.4748344903314));
#40577=CARTESIAN_POINT('Ctrl Pts',(-16.3387721302027,18.3074052613332,-13.4792209523439));
#40578=CARTESIAN_POINT('Ctrl Pts',(-16.3682848706079,18.229173577031,-13.4834055867369));
#40579=CARTESIAN_POINT('Ctrl Pts',(-16.4016893071736,18.1522437219302,-13.48759022113));
#40580=CARTESIAN_POINT('Ctrl Pts',(-16.4388502681124,18.0770301114156,-13.491774855523));
#40581=CARTESIAN_POINT('Ctrl Pts',(-16.4759583350228,18.0019235581661,-13.495953533607));
#40582=CARTESIAN_POINT('Ctrl Pts',(-16.5168121035541,17.9285288061221,-13.5001322116909));
#40583=CARTESIAN_POINT('Ctrl Pts',(-16.5612276601908,17.8572421341466,-13.5043108897749));
#40584=CARTESIAN_POINT('Ctrl Pts',(-16.6064393337593,17.7846776998087,-13.5085644676603));
#40585=CARTESIAN_POINT('Ctrl Pts',(-16.6553415713116,17.7142981146653,-13.5128180455457));
#40586=CARTESIAN_POINT('Ctrl Pts',(-16.7076904562346,17.6464970013307,-13.5170716234312));
#40587=CARTESIAN_POINT('Ctrl Pts',(-16.7590244558731,17.580010344881,-13.5212427374091));
#40588=CARTESIAN_POINT('Ctrl Pts',(-16.8136723614031,17.5160034559041,-13.5254138513871));
#40589=CARTESIAN_POINT('Ctrl Pts',(-16.8713604260513,17.4548183984679,-13.529584965365));
#40590=CARTESIAN_POINT('Ctrl Pts',(-16.9290291329122,17.3936538722685,-13.5337546796854));
#40591=CARTESIAN_POINT('Ctrl Pts',(-16.9897356575239,17.3353096315042,-13.5379243940058));
#40592=CARTESIAN_POINT('Ctrl Pts',(-17.0531673758219,17.2800930396577,-13.5420941083262));
#40593=CARTESIAN_POINT('Ctrl Pts',(-17.116596836947,17.2248784126545,-13.5462636742702));
#40594=CARTESIAN_POINT('Ctrl Pts',(-17.1827509514049,17.172791514689,-13.5504332402142));
#40595=CARTESIAN_POINT('Ctrl Pts',(-17.2512828336366,17.1241004325624,-13.5546028061583));
#40596=CARTESIAN_POINT('Ctrl Pts',(-17.3222242123044,17.0736974320551,-13.5589189688972));
#40597=CARTESIAN_POINT('Ctrl Pts',(-17.395713244423,17.0269337896177,-13.5632351316361));
#40598=CARTESIAN_POINT('Ctrl Pts',(-17.4713327209557,16.98405784933,-13.567551294375));
#40599=CARTESIAN_POINT('Ctrl Pts',(-17.5444889009941,16.9425785882874,-13.5717268585667));
#40600=CARTESIAN_POINT('Ctrl Pts',(-17.6196384165434,16.9047378049044,-13.5759024227584));
#40601=CARTESIAN_POINT('Ctrl Pts',(-17.6963803894308,16.8707125083097,-13.5800779869501));
#40602=CARTESIAN_POINT('Ctrl Pts',(-17.7769984169321,16.8349686748714,-13.5844644489626));
#40603=CARTESIAN_POINT('Ctrl Pts',(-17.8593734542574,16.8034361069936,-13.5888509109752));
#40604=CARTESIAN_POINT('Ctrl Pts',(-17.9430216212717,16.7762611630024,-13.5932373729877));
#40605=CARTESIAN_POINT('Ctrl Pts',(-18.026669788286,16.7490862190113,-13.5976238350002));
#40606=CARTESIAN_POINT('Ctrl Pts',(-18.1115905049086,16.726268976005,-13.6020102970128));
#40607=CARTESIAN_POINT('Ctrl Pts',(-18.1972887614196,16.7078937205182,-13.6063967590253));
#40608=CARTESIAN_POINT('Ctrl Pts',(-18.2790439141132,16.6903639377749,-13.6105813934184));
#40609=CARTESIAN_POINT('Ctrl Pts',(-18.3618109357872,16.6768111110841,-13.6147660278114));
#40610=CARTESIAN_POINT('Ctrl Pts',(-18.4451682027608,16.6673458975514,-13.6189506622045));
#40611=CARTESIAN_POINT('Ctrl Pts',(-18.5284068209825,16.6578941565786,-13.6231293402884));
#40612=CARTESIAN_POINT('Ctrl Pts',(-18.6122335625331,16.6525185234246,-13.6273080183724));
#40613=CARTESIAN_POINT('Ctrl Pts',(-18.696215670704,16.6512788541602,-13.6314866964563));
#40614=CARTESIAN_POINT('Ctrl Pts',(-18.7817030978069,16.6500169647151,-13.6357402743417));
#40615=CARTESIAN_POINT('Ctrl Pts',(-18.8673510447845,16.6530408729659,-13.6399938522272));
#40616=CARTESIAN_POINT('Ctrl Pts',(-18.9526965098738,16.6603585440974,-13.6442474301126));
#40617=CARTESIAN_POINT('Ctrl Pts',(-19.0363873865844,16.6675343478947,-13.6484185440906));
#40618=CARTESIAN_POINT('Ctrl Pts',(-19.1197869256881,16.6788388732104,-13.6525896580685));
#40619=CARTESIAN_POINT('Ctrl Pts',(-19.2024593315,16.6942270951215,-13.6567607720465));
#40620=CARTESIAN_POINT('Ctrl Pts',(-19.2851039957877,16.7096101533661,-13.6609304863668));
#40621=CARTESIAN_POINT('Ctrl Pts',(-19.3670215594762,16.7290741026091,-13.6651002006872));
#40622=CARTESIAN_POINT('Ctrl Pts',(-19.4477843610411,16.7525224455096,-13.6692699150076));
#40623=CARTESIAN_POINT('Ctrl Pts',(-19.5285442887189,16.7759699540174,-13.6734394809516));
#40624=CARTESIAN_POINT('Ctrl Pts',(-19.6081490944216,16.8034014451984,-13.6776090468957));
#40625=CARTESIAN_POINT('Ctrl Pts',(-19.6861855970015,16.8346703534941,-13.6817786128397));
#40626=CARTESIAN_POINT('Ctrl Pts',(-19.7669657667436,16.8670386380311,-13.6860947755787));
#40627=CARTESIAN_POINT('Ctrl Pts',(-19.8460648087827,16.9035190114426,-13.6904109383176));
#40628=CARTESIAN_POINT('Ctrl Pts',(-19.9230480777103,16.9438950908938,-13.6947271010565));
#40629=CARTESIAN_POINT('Ctrl Pts',(-19.9975236247499,16.9829559238037,-13.6989026652482));
#40630=CARTESIAN_POINT('Ctrl Pts',(-20.0700187425847,17.025662275374,-13.7030782294399));
#40631=CARTESIAN_POINT('Ctrl Pts',(-20.1401676067983,17.0717728821859,-13.7072537936315));
#40632=CARTESIAN_POINT('Ctrl Pts',(-20.2138595233803,17.1202124261303,-13.7116402556441));
#40633=CARTESIAN_POINT('Ctrl Pts',(-20.2849614681664,17.1724088154589,-13.7160267176566));
#40634=CARTESIAN_POINT('Ctrl Pts',(-20.3530884618268,17.2280344045396,-13.7204131796692));
#40635=CARTESIAN_POINT('Ctrl Pts',(-20.4212154554871,17.2836599936204,-13.7247996416817));
#40636=CARTESIAN_POINT('Ctrl Pts',(-20.4863671192074,17.3427143364292,-13.7291861036943));
#40637=CARTESIAN_POINT('Ctrl Pts',(-20.548204641978,17.4048268308311,-13.7335725657068));
#40638=CARTESIAN_POINT('Ctrl Pts',(-20.6067777194386,17.4636603639817,-13.7377274633762));
#40639=CARTESIAN_POINT('Ctrl Pts',(-20.6626103382647,17.5254713783546,-13.7418823610455));
#40640=CARTESIAN_POINT('Ctrl Pts',(-20.7153787245625,17.5899699725634,-13.7460372587149));
#40641=CARTESIAN_POINT('Ctrl Pts',(-20.7677053791601,17.6539286398258,-13.7501573751423));
#40642=CARTESIAN_POINT('Ctrl Pts',(-20.8170185699061,17.7205297194409,-13.7542774915697));
#40643=CARTESIAN_POINT('Ctrl Pts',(-20.8630375889925,17.7894519196816,-13.7583976079971));
#40644=CARTESIAN_POINT('Ctrl Pts',(-20.9090125260321,17.8583080987051,-13.7625137777266));
#40645=CARTESIAN_POINT('Ctrl Pts',(-20.951699290088,17.9294805955782,-13.7666299474561));
#40646=CARTESIAN_POINT('Ctrl Pts',(-20.9908578231797,18.0026156381546,-13.7707461171856));
#40647=CARTESIAN_POINT('Ctrl Pts',(-21.0299913601116,18.0757039962649,-13.7748596594307));
#40648=CARTESIAN_POINT('Ctrl Pts',(-21.0656009133711,18.1507519968574,-13.7789732016758));
#40649=CARTESIAN_POINT('Ctrl Pts',(-21.0974909394082,18.2273788435911,-13.7830867439209));
#40650=CARTESIAN_POINT('Ctrl Pts',(-21.1299241917558,18.3053109799219,-13.7872703577417));
#40651=CARTESIAN_POINT('Ctrl Pts',(-21.1585097661409,18.3848758167557,-13.7914539715626));
#40652=CARTESIAN_POINT('Ctrl Pts',(-21.1830923574767,18.4656499986255,-13.7956375853835));
#40653=CARTESIAN_POINT('Ctrl Pts',(-21.2072638620762,18.5450734199364,-13.7997512379815));
#40654=CARTESIAN_POINT('Ctrl Pts',(-21.2275651518659,18.6256655681997,-13.8038648905795));
#40655=CARTESIAN_POINT('Ctrl Pts',(-21.2438990336338,18.7070090864272,-13.8079785431775));
#40656=CARTESIAN_POINT('Ctrl Pts',(-21.260649602877,18.7904277283589,-13.8121971376098));
#40657=CARTESIAN_POINT('Ctrl Pts',(-21.2732274574716,18.8746360871023,-13.8164157320421));
#40658=CARTESIAN_POINT('Ctrl Pts',(-21.2815840465261,18.9591756050627,-13.8206343264745));
#40659=CARTESIAN_POINT('Ctrl Pts',(-21.2899406355806,19.043715123023,-13.8248529209068));
#40660=CARTESIAN_POINT('Ctrl Pts',(-21.2940759677847,19.1285852645553,-13.8290715153392));
#40661=CARTESIAN_POINT('Ctrl Pts',(-21.2939989424941,19.2133268925441,-13.8332901097715));
#40662=CARTESIAN_POINT('Ctrl Pts',(-21.2944497455462,19.2133273022983,-13.8332901097715));
#40663=CARTESIAN_POINT('Ctrl Pts',(-21.2961552640167,19.3972186594194,-13.8424428639771));
#40664=CARTESIAN_POINT('Ctrl Pts',(-21.1940977855363,20.4309438993384,-13.8939875537431));
#40665=CARTESIAN_POINT('Ctrl Pts',(-19.7898863418736,22.047969473252,-13.9879241790696));
#40666=CARTESIAN_POINT('Ctrl Pts',(-17.8646300978083,21.7705396626413,-14.0732424008125));
#40667=CARTESIAN_POINT('Ctrl Pts',(-17.1803677633157,21.2509974006736,-14.1161686869948));
#40668=CARTESIAN_POINT('Ctrl Pts',(-17.1718944362858,21.2444720185936,-14.1167030376167));
#40669=CARTESIAN_POINT('',(-21.2939989173812,19.2086456408557,-13.7667098774912));
#40670=CARTESIAN_POINT('Ctrl Pts',(-21.2935817003363,19.2086462806877,-13.7667098902285));
#40671=CARTESIAN_POINT('Ctrl Pts',(-21.2877698482561,19.8484613719781,-13.7985275695778));
#40672=CARTESIAN_POINT('Ctrl Pts',(-20.7208250258792,21.3499116215441,-13.8727371844875));
#40673=CARTESIAN_POINT('Ctrl Pts',(-18.6774627206427,22.0308987559626,-13.9672098138401));
#40674=CARTESIAN_POINT('Ctrl Pts',(-17.5010449849498,21.4873580244075,-14.0298647638434));
#40675=CARTESIAN_POINT('Ctrl Pts',(-17.1770151058749,21.2378231662188,-14.0501277782861));
#40676=CARTESIAN_POINT('Ctrl Pts',(-17.1744642439897,21.2411350264762,-13.2501880045741));
#40677=CARTESIAN_POINT('Ctrl Pts',(-17.1058906060324,21.1884572297191,-13.2544909919482));
#40678=CARTESIAN_POINT('Ctrl Pts',(-17.0399076063725,21.1322386433023,-13.2587939793222));
#40679=CARTESIAN_POINT('Ctrl Pts',(-16.9768963495314,21.0727697928342,-13.2630969666962));
#40680=CARTESIAN_POINT('Ctrl Pts',(-16.9158136728346,21.0151211003818,-13.267268252904));
#40681=CARTESIAN_POINT('Ctrl Pts',(-16.8575238163474,20.9544185704731,-13.2714395391118));
#40682=CARTESIAN_POINT('Ctrl Pts',(-16.8023406084374,20.8909678553436,-13.2756108253196));
#40683=CARTESIAN_POINT('Ctrl Pts',(-16.7471772900096,20.827540009524,-13.279780608086));
#40684=CARTESIAN_POINT('Ctrl Pts',(-16.6951186980832,20.7613662923708,-13.2839503908523));
#40685=CARTESIAN_POINT('Ctrl Pts',(-16.6464403664802,20.6927876961625,-13.2881201736186));
#40686=CARTESIAN_POINT('Ctrl Pts',(-16.5977649775094,20.6242132455685,-13.2922897043193));
#40687=CARTESIAN_POINT('Ctrl Pts',(-16.552469708406,20.5532345804094,-13.2964592350199));
#40688=CARTESIAN_POINT('Ctrl Pts',(-16.5107876884942,20.4802229977308,-13.3006287657206));
#40689=CARTESIAN_POINT('Ctrl Pts',(-16.469095684905,20.4071939273181,-13.3047992951072));
#40690=CARTESIAN_POINT('Ctrl Pts',(-16.4310188759036,20.3321313725595,-13.3089698244939));
#40691=CARTESIAN_POINT('Ctrl Pts',(-16.3967445544524,20.2554314157751,-13.3131403538805));
#40692=CARTESIAN_POINT('Ctrl Pts',(-16.3624311523989,20.1786440034151,-13.317315638629));
#40693=CARTESIAN_POINT('Ctrl Pts',(-16.3319290757362,20.1002158846929,-13.3214909233775));
#40694=CARTESIAN_POINT('Ctrl Pts',(-16.3053773193722,20.0205627678817,-13.325666208126));
#40695=CARTESIAN_POINT('Ctrl Pts',(-16.2788073074776,19.9408548859585,-13.3298443635711));
#40696=CARTESIAN_POINT('Ctrl Pts',(-16.2561931439568,19.8599207723268,-13.3340225190163));
#40697=CARTESIAN_POINT('Ctrl Pts',(-16.2376232149648,19.7781886345276,-13.3382006744614));
#40698=CARTESIAN_POINT('Ctrl Pts',(-16.2190239845482,19.6963275318802,-13.3423854226031));
#40699=CARTESIAN_POINT('Ctrl Pts',(-16.2044817977587,19.6136663447483,-13.3465701707449));
#40700=CARTESIAN_POINT('Ctrl Pts',(-16.1940334279964,19.5306401306222,-13.3507549188866));
#40701=CARTESIAN_POINT('Ctrl Pts',(-16.191782351114,19.5127523265437,-13.3516565131079));
#40702=CARTESIAN_POINT('Ctrl Pts',(-16.1897211074132,19.4948475818153,-13.3525581073293));
#40703=CARTESIAN_POINT('Ctrl Pts',(-16.1878497481282,19.4769302444118,-13.3534597015506));
#40704=CARTESIAN_POINT('Ctrl Pts',(-16.1791640730867,19.3937692119263,-13.3576443359437));
#40705=CARTESIAN_POINT('Ctrl Pts',(-16.1745407622114,19.3100274422731,-13.3618289703367));
#40706=CARTESIAN_POINT('Ctrl Pts',(-16.1740447460464,19.2261359755289,-13.3660136047298));
#40707=CARTESIAN_POINT('Ctrl Pts',(-16.173549435899,19.1423639179039,-13.3701922828137));
#40708=CARTESIAN_POINT('Ctrl Pts',(-16.1771697541693,19.0584430425126,-13.3743709608977));
#40709=CARTESIAN_POINT('Ctrl Pts',(-16.1849189310737,18.9748100255276,-13.3785496389816));
#40710=CARTESIAN_POINT('Ctrl Pts',(-16.1928070064048,18.8896779468192,-13.382803216867));
#40711=CARTESIAN_POINT('Ctrl Pts',(-16.2049734659499,18.804844627276,-13.3870567947525));
#40712=CARTESIAN_POINT('Ctrl Pts',(-16.2213767120001,18.7207712650195,-13.3913103726379));
#40713=CARTESIAN_POINT('Ctrl Pts',(-16.2374619491174,18.6383278289459,-13.3954814866159));
#40714=CARTESIAN_POINT('Ctrl Pts',(-16.2576210698179,18.5566156189164,-13.3996526005938));
#40715=CARTESIAN_POINT('Ctrl Pts',(-16.2817626998464,18.4760631158151,-13.4038237145718));
#40716=CARTESIAN_POINT('Ctrl Pts',(-16.3058962289179,18.3955376428842,-13.4079934288921));
#40717=CARTESIAN_POINT('Ctrl Pts',(-16.3340094813079,18.3161715443229,-13.4121631432125));
#40718=CARTESIAN_POINT('Ctrl Pts',(-16.3659607754927,18.2383797086247,-13.4163328575329));
#40719=CARTESIAN_POINT('Ctrl Pts',(-16.3979109327134,18.1605906410939,-13.4205024234769));
#40720=CARTESIAN_POINT('Ctrl Pts',(-16.4336986846161,18.0843761502596,-13.424671989421));
#40721=CARTESIAN_POINT('Ctrl Pts',(-16.4731341172713,18.0101313725834,-13.428841555365));
#40722=CARTESIAN_POINT('Ctrl Pts',(-16.5139560510898,17.933276240115,-13.433157718104));
#40723=CARTESIAN_POINT('Ctrl Pts',(-16.5586866956794,17.8585323739429,-13.4374738808429));
#40724=CARTESIAN_POINT('Ctrl Pts',(-16.6070644247003,17.7863087848504,-13.4417900435818));
#40725=CARTESIAN_POINT('Ctrl Pts',(-16.6538662542868,17.7164378715759,-13.4459656077735));
#40726=CARTESIAN_POINT('Ctrl Pts',(-16.7040808906405,17.6489259106341,-13.4501411719652));
#40727=CARTESIAN_POINT('Ctrl Pts',(-16.7574293298199,17.5841108255988,-13.4543167361568));
#40728=CARTESIAN_POINT('Ctrl Pts',(-16.8134722718384,17.5160220847016,-13.4587031981694));
#40729=CARTESIAN_POINT('Ctrl Pts',(-16.8729735193545,17.450910248947,-13.4630896601819));
#40730=CARTESIAN_POINT('Ctrl Pts',(-16.9355661330671,17.3891230485379,-13.4674761221945));
#40731=CARTESIAN_POINT('Ctrl Pts',(-16.9981587467797,17.3273358481289,-13.471862584207));
#40732=CARTESIAN_POINT('Ctrl Pts',(-17.0638422427094,17.2688736120054,-13.4762490462195));
#40733=CARTESIAN_POINT('Ctrl Pts',(-17.1322119090441,17.2140335727229,-13.4806355082321));
#40734=CARTESIAN_POINT('Ctrl Pts',(-17.1974357856826,17.1617168049403,-13.4848201426251));
#40735=CARTESIAN_POINT('Ctrl Pts',(-17.2653468510498,17.112501500524,-13.4890047770182));
#40736=CARTESIAN_POINT('Ctrl Pts',(-17.3356178143268,17.0666755696043,-13.4931894114112));
#40737=CARTESIAN_POINT('Ctrl Pts',(-17.4057887555853,17.0209148662252,-13.4973680894952));
#40738=CARTESIAN_POINT('Ctrl Pts',(-17.4783125406378,16.9785342027988,-13.5015467675791));
#40739=CARTESIAN_POINT('Ctrl Pts',(-17.5528291551938,16.9397810683732,-13.5057254456631));
#40740=CARTESIAN_POINT('Ctrl Pts',(-17.6286814265116,16.9003333118645,-13.5099790235485));
#40741=CARTESIAN_POINT('Ctrl Pts',(-17.7065982968802,16.8646447120803,-13.5142326014339));
#40742=CARTESIAN_POINT('Ctrl Pts',(-17.7861694556147,16.8329299297266,-13.5184861793194));
#40743=CARTESIAN_POINT('Ctrl Pts',(-17.8641979721668,16.8018300003151,-13.5226572932973));
#40744=CARTESIAN_POINT('Ctrl Pts',(-17.9438167592513,16.7745513610798,-13.5268284072753));
#40745=CARTESIAN_POINT('Ctrl Pts',(-18.0246160731017,16.7512491093084,-13.5309995212532));
#40746=CARTESIAN_POINT('Ctrl Pts',(-18.105388273962,16.7279546768326,-13.5351692355736));
#40747=CARTESIAN_POINT('Ctrl Pts',(-18.1873397732034,16.7086341092198,-13.539338949894));
#40748=CARTESIAN_POINT('Ctrl Pts',(-18.2700450257387,16.6933928460027,-13.5435086642143));
#40749=CARTESIAN_POINT('Ctrl Pts',(-18.3527473352662,16.6781521251352,-13.5476782301584));
#40750=CARTESIAN_POINT('Ctrl Pts',(-18.4362028921897,16.6669905025844,-13.5518477961024));
#40751=CARTESIAN_POINT('Ctrl Pts',(-18.5199766524687,16.6599621706624,-13.5560173620465));
#40752=CARTESIAN_POINT('Ctrl Pts',(-18.606695794813,16.6526867312604,-13.5603335247854));
#40753=CARTESIAN_POINT('Ctrl Pts',(-18.693755407323,16.6498406874529,-13.5646496875243));
#40754=CARTESIAN_POINT('Ctrl Pts',(-18.7806699632819,16.6514254426708,-13.5689658502632));
#40755=CARTESIAN_POINT('Ctrl Pts',(-18.8647532867223,16.6529585746541,-13.5731414144549));
#40756=CARTESIAN_POINT('Ctrl Pts',(-18.9487003921372,16.6586381931969,-13.5773169786466));
#40757=CARTESIAN_POINT('Ctrl Pts',(-19.032076119737,16.6684126117589,-13.5814925428383));
#40758=CARTESIAN_POINT('Ctrl Pts',(-19.1196629571308,16.6786807129661,-13.5858790048508));
#40759=CARTESIAN_POINT('Ctrl Pts',(-19.2066186035791,16.6934680441002,-13.5902654668633));
#40760=CARTESIAN_POINT('Ctrl Pts',(-19.2924520557265,16.7126542870422,-13.5946519288759));
#40761=CARTESIAN_POINT('Ctrl Pts',(-19.3782855078739,16.7318405299841,-13.5990383908884));
#40762=CARTESIAN_POINT('Ctrl Pts',(-19.462996227165,16.7554254558327,-13.603424852901));
#40763=CARTESIAN_POINT('Ctrl Pts',(-19.5461152252309,16.783229652346,-13.6078113149135));
#40764=CARTESIAN_POINT('Ctrl Pts',(-19.6254097949838,16.809754536562,-13.6119959493065));
#40765=CARTESIAN_POINT('Ctrl Pts',(-19.7035510491552,16.8402176845382,-13.6161805836996));
#40766=CARTESIAN_POINT('Ctrl Pts',(-19.7801197445754,16.8744997367838,-13.6203652180926));
#40767=CARTESIAN_POINT('Ctrl Pts',(-19.856579453935,16.9087329927713,-13.6245438961766));
#40768=CARTESIAN_POINT('Ctrl Pts',(-19.9314706343179,16.9467741695628,-13.6287225742605));
#40769=CARTESIAN_POINT('Ctrl Pts',(-20.0043903176931,16.9884545132413,-13.6329012523445));
#40770=CARTESIAN_POINT('Ctrl Pts',(-20.0786170339864,17.0308819471251,-13.6371548302299));
#40771=CARTESIAN_POINT('Ctrl Pts',(-20.1508004226817,17.0770801423177,-13.6414084081153));
#40772=CARTESIAN_POINT('Ctrl Pts',(-20.2205378947047,17.1268202842349,-13.6456619860008));
#40773=CARTESIAN_POINT('Ctrl Pts',(-20.288923369751,17.1755961164411,-13.6498330999787));
#40774=CARTESIAN_POINT('Ctrl Pts',(-20.3549565277687,17.2277775063951,-13.6540042139567));
#40775=CARTESIAN_POINT('Ctrl Pts',(-20.4182851699542,17.283103875653,-13.6581753279346));
#40776=CARTESIAN_POINT('Ctrl Pts',(-20.4815925616022,17.3384116796133,-13.662345042255));
#40777=CARTESIAN_POINT('Ctrl Pts',(-20.5421968936246,17.3968620645641,-13.6665147565753));
#40778=CARTESIAN_POINT('Ctrl Pts',(-20.5997791685761,17.4581542868503,-13.6706844708957));
#40779=CARTESIAN_POINT('Ctrl Pts',(-20.6573593945032,17.5194443280962,-13.6748540368398));
#40780=CARTESIAN_POINT('Ctrl Pts',(-20.7119174628062,17.5835756697508,-13.6790236027838));
#40781=CARTESIAN_POINT('Ctrl Pts',(-20.763172325239,17.6502118418939,-13.6831931687278));
#40782=CARTESIAN_POINT('Ctrl Pts',(-20.8162292454052,17.719190859645,-13.6875093314668));
#40783=CARTESIAN_POINT('Ctrl Pts',(-20.8657460348867,17.79085370675,-13.6918254942057));
#40784=CARTESIAN_POINT('Ctrl Pts',(-20.911458707217,17.864792891727,-13.6961416569446));
#40785=CARTESIAN_POINT('Ctrl Pts',(-20.9556822940543,17.9363235155303,-13.7003172211363));
#40786=CARTESIAN_POINT('Ctrl Pts',(-20.9963456096572,18.0099840160616,-13.704492785328));
#40787=CARTESIAN_POINT('Ctrl Pts',(-21.0332565704859,18.0853805158591,-13.7086683495196));
#40788=CARTESIAN_POINT('Ctrl Pts',(-21.0720318161985,18.1645851136233,-13.7130548115322));
#40789=CARTESIAN_POINT('Ctrl Pts',(-21.1066654530387,18.245705153136,-13.7174412735447));
#40790=CARTESIAN_POINT('Ctrl Pts',(-21.1369928787006,18.3282626523623,-13.7218277355573));
#40791=CARTESIAN_POINT('Ctrl Pts',(-21.1673203043624,18.4108201515887,-13.7262141975698));
#40792=CARTESIAN_POINT('Ctrl Pts',(-21.1933414198056,18.494814533789,-13.7306006595824));
#40793=CARTESIAN_POINT('Ctrl Pts',(-21.214953227824,18.5797543415201,-13.7349871215949));
#40794=CARTESIAN_POINT('Ctrl Pts',(-21.2416966549181,18.6848626949492,-13.740415127754));
#40795=CARTESIAN_POINT('Ctrl Pts',(-21.2617718479477,18.7917315462695,-13.7458431339131));
#40796=CARTESIAN_POINT('Ctrl Pts',(-21.2749934581325,18.8996284442541,-13.7512711400722));
#40797=CARTESIAN_POINT('Ctrl Pts',(-21.2875287526721,19.0019245622934,-13.7564173858785));
#40798=CARTESIAN_POINT('Ctrl Pts',(-21.2939037306914,19.1051449394058,-13.7615636316849));
#40799=CARTESIAN_POINT('Ctrl Pts',(-21.2939989173812,19.2086456408557,-13.7667098774912));
#40800=CARTESIAN_POINT('Origin',(-18.734,19.211,1.76670989022852));
#40801=CARTESIAN_POINT('',(-17.1725834302249,21.2436206685575,-12.4500366781978));
#40802=CARTESIAN_POINT('',(-17.1744642439897,21.2411350264762,-12.5167193432124));
#40803=CARTESIAN_POINT('',(-17.1744642439897,21.2411350264762,1.76670989022852));
#40804=CARTESIAN_POINT('',(-21.293999998394,19.2109093211998,-13.0332901097364));
#40805=CARTESIAN_POINT('Ctrl Pts',(-17.1744642439897,21.2411350264762,-12.5167193432124));
#40806=CARTESIAN_POINT('Ctrl Pts',(-17.1077874800253,21.1899143952662,-12.5208888590638));
#40807=CARTESIAN_POINT('Ctrl Pts',(-17.0436201898523,21.1353927403986,-12.5250583749152));
#40808=CARTESIAN_POINT('Ctrl Pts',(-16.9822976161262,21.077852634337,-12.5292278907666));
#40809=CARTESIAN_POINT('Ctrl Pts',(-16.9209705475262,21.0203083106519,-12.5333977122387));
#40810=CARTESIAN_POINT('Ctrl Pts',(-16.8624889439855,20.9597454121972,-12.5375675337108));
#40811=CARTESIAN_POINT('Ctrl Pts',(-16.8071520646769,20.8964842135544,-12.5417373551829));
#40812=CARTESIAN_POINT('Ctrl Pts',(-16.7517573571547,20.833156905616,-12.545911534207));
#40813=CARTESIAN_POINT('Ctrl Pts',(-16.6995142397073,20.7671260137235,-12.550085713231));
#40814=CARTESIAN_POINT('Ctrl Pts',(-16.6506820992389,20.6987454501252,-12.5542598922551));
#40815=CARTESIAN_POINT('Ctrl Pts',(-16.6018236631547,20.6303280642822,-12.5584363190325));
#40816=CARTESIAN_POINT('Ctrl Pts',(-16.5563801103552,20.559558874473,-12.5626127458099));
#40817=CARTESIAN_POINT('Ctrl Pts',(-16.5145664970211,20.4868193155203,-12.5667891725874));
#40818=CARTESIAN_POINT('Ctrl Pts',(-16.4726800356492,20.4139530290807,-12.5709728755716));
#40819=CARTESIAN_POINT('Ctrl Pts',(-16.4344363552231,20.3391099268244,-12.5751565785557));
#40820=CARTESIAN_POINT('Ctrl Pts',(-16.400003615296,20.2626942883692,-12.5793402815399));
#40821=CARTESIAN_POINT('Ctrl Pts',(-16.3735297181201,20.2039414920662,-12.5825569562179));
#40822=CARTESIAN_POINT('Ctrl Pts',(-16.3493076693354,20.1442595816972,-12.5857736308959));
#40823=CARTESIAN_POINT('Ctrl Pts',(-16.3273937923111,20.0838382216157,-12.5889903055739));
#40824=CARTESIAN_POINT('Ctrl Pts',(-16.2988856052357,20.0052349039716,-12.5931749399669));
#40825=CARTESIAN_POINT('Ctrl Pts',(-16.274179366091,19.9250871608004,-12.59735957436));
#40826=CARTESIAN_POINT('Ctrl Pts',(-16.2534421603042,19.8437976010729,-12.601544208753));
#40827=CARTESIAN_POINT('Ctrl Pts',(-16.2327344713631,19.7626237469723,-12.605722886837));
#40828=CARTESIAN_POINT('Ctrl Pts',(-16.2159847069801,19.680311746487,-12.6099015649209));
#40829=CARTESIAN_POINT('Ctrl Pts',(-16.2033111427938,19.5972821611364,-12.6140802430048));
#40830=CARTESIAN_POINT('Ctrl Pts',(-16.1904104140777,19.5127643301405,-12.6183338208903));
#40831=CARTESIAN_POINT('Ctrl Pts',(-16.1817336190672,19.4275033890776,-12.6225873987757));
#40832=CARTESIAN_POINT('Ctrl Pts',(-16.177351748603,19.3419569342513,-12.6268409766612));
#40833=CARTESIAN_POINT('Ctrl Pts',(-16.1730548292483,19.2580689643821,-12.6310120906391));
#40834=CARTESIAN_POINT('Ctrl Pts',(-16.1728878141637,19.1739069330302,-12.6351832046171));
#40835=CARTESIAN_POINT('Ctrl Pts',(-16.1768654907269,19.0899087059925,-12.639354318595));
#40836=CARTESIAN_POINT('Ctrl Pts',(-16.1808418325422,19.0059386653711,-12.6435240329154));
#40837=CARTESIAN_POINT('Ctrl Pts',(-16.1889600821296,18.922132779036,-12.6476937472358));
#40838=CARTESIAN_POINT('Ctrl Pts',(-16.2011829261396,18.8389278694111,-12.6518634615561));
#40839=CARTESIAN_POINT('Ctrl Pts',(-16.2134053352083,18.7557259205741,-12.6560330275002));
#40840=CARTESIAN_POINT('Ctrl Pts',(-16.229731980592,18.673125360952,-12.6602025934442));
#40841=CARTESIAN_POINT('Ctrl Pts',(-16.250073974422,18.5915554912213,-12.6643721593882));
#40842=CARTESIAN_POINT('Ctrl Pts',(-16.2711311676605,18.5071177254979,-12.6686883221272));
#40843=CARTESIAN_POINT('Ctrl Pts',(-16.2964911945896,18.4237849880538,-12.6730044848661));
#40844=CARTESIAN_POINT('Ctrl Pts',(-16.325998926724,18.3420173585728,-12.677320647605));
#40845=CARTESIAN_POINT('Ctrl Pts',(-16.3545454475878,18.2629133010219,-12.6814962117967));
#40846=CARTESIAN_POINT('Ctrl Pts',(-16.3869733753121,18.1852743669885,-12.6856717759884));
#40847=CARTESIAN_POINT('Ctrl Pts',(-16.4230935537342,18.1094958481209,-12.6898473401801));
#40848=CARTESIAN_POINT('Ctrl Pts',(-16.4610380765009,18.0298899364114,-12.6942338021926));
#40849=CARTESIAN_POINT('Ctrl Pts',(-16.5030573653642,17.9523378315092,-12.6986202642051));
#40850=CARTESIAN_POINT('Ctrl Pts',(-16.5488792984353,17.8772655738142,-12.7030067262177));
#40851=CARTESIAN_POINT('Ctrl Pts',(-16.5947012315064,17.8021933161192,-12.7073931882302));
#40852=CARTESIAN_POINT('Ctrl Pts',(-16.6443254185491,17.7296013416972,-12.7117796502428));
#40853=CARTESIAN_POINT('Ctrl Pts',(-16.6974308899397,17.6598758076968,-12.7161661122553));
#40854=CARTESIAN_POINT('Ctrl Pts',(-16.7480928998703,17.593358448874,-12.7203507466484));
#40855=CARTESIAN_POINT('Ctrl Pts',(-16.8021114495637,17.5292019583441,-12.7245353810414));
#40856=CARTESIAN_POINT('Ctrl Pts',(-16.8592384487626,17.4677647531094,-12.7287200154345));
#40857=CARTESIAN_POINT('Ctrl Pts',(-16.9162841347489,17.4064149961321,-12.7328986935184));
#40858=CARTESIAN_POINT('Ctrl Pts',(-16.9764291712243,17.3477771703016,-12.7370773716023));
#40859=CARTESIAN_POINT('Ctrl Pts',(-17.0393839528664,17.2921783686863,-12.7412560496863));
#40860=CARTESIAN_POINT('Ctrl Pts',(-17.1034671537248,17.2355829985101,-12.7455096275717));
#40861=CARTESIAN_POINT('Ctrl Pts',(-17.1704615277515,17.1821370567432,-12.7497632054571));
#40862=CARTESIAN_POINT('Ctrl Pts',(-17.2400207348668,17.1321479236482,-12.7540167833426));
#40863=CARTESIAN_POINT('Ctrl Pts',(-17.3082314010186,17.0831279274441,-12.7581878973205));
#40864=CARTESIAN_POINT('Ctrl Pts',(-17.3789079483578,17.0374321828771,-12.7623590112985));
#40865=CARTESIAN_POINT('Ctrl Pts',(-17.4516902051699,16.9953101322426,-12.7665301252764));
#40866=CARTESIAN_POINT('Ctrl Pts',(-17.5244480391927,16.9532022160691,-12.7706998395968));
#40867=CARTESIAN_POINT('Ctrl Pts',(-17.5993097815583,16.9146658424624,-12.7748695539171));
#40868=CARTESIAN_POINT('Ctrl Pts',(-17.6758879367283,16.8799060804938,-12.7790392682375));
#40869=CARTESIAN_POINT('Ctrl Pts',(-17.7524633669187,16.8451475554268,-12.7832088341815));
#40870=CARTESIAN_POINT('Ctrl Pts',(-17.8307546692255,16.814165564167,-12.7873784001256));
#40871=CARTESIAN_POINT('Ctrl Pts',(-17.9103527564008,16.7871177383975,-12.7915479660696));
#40872=CARTESIAN_POINT('Ctrl Pts',(-17.9927494141267,16.7591189444408,-12.7958641288085));
#40873=CARTESIAN_POINT('Ctrl Pts',(-18.0765459602113,16.7353362835288,-12.8001802915474));
#40874=CARTESIAN_POINT('Ctrl Pts',(-18.1612715723428,16.7158883495616,-12.8044964542864));
#40875=CARTESIAN_POINT('Ctrl Pts',(-18.2432372565706,16.6970739299979,-12.808672018478));
#40876=CARTESIAN_POINT('Ctrl Pts',(-18.3260719356978,16.6823162029297,-12.8128475826697));
#40877=CARTESIAN_POINT('Ctrl Pts',(-18.4093408453614,16.6716700818308,-12.8170231468614));
#40878=CARTESIAN_POINT('Ctrl Pts',(-18.4968154696991,16.6604862504638,-12.8214096088739));
#40879=CARTESIAN_POINT('Ctrl Pts',(-18.584768761138,16.6538403392096,-12.8257960708865));
#40880=CARTESIAN_POINT('Ctrl Pts',(-18.6726951927067,16.6517341442119,-12.830182532899));
#40881=CARTESIAN_POINT('Ctrl Pts',(-18.7606216242755,16.6496279492142,-12.8345689949116));
#40882=CARTESIAN_POINT('Ctrl Pts',(-18.8485206180843,16.6520613783803,-12.8389554569241));
#40883=CARTESIAN_POINT('Ctrl Pts',(-18.9358937423124,16.6589735665916,-12.8433419189367));
#40884=CARTESIAN_POINT('Ctrl Pts',(-19.0192466995765,16.665567714777,-12.8475265533297));
#40885=CARTESIAN_POINT('Ctrl Pts',(-19.1024313715336,16.6762620749485,-12.8517111877228));
#40886=CARTESIAN_POINT('Ctrl Pts',(-19.1850120996546,16.6910420467863,-12.8558958221158));
#40887=CARTESIAN_POINT('Ctrl Pts',(-19.2674752843308,16.7058009811636,-12.8600745001998));
#40888=CARTESIAN_POINT('Ctrl Pts',(-19.3493357837208,16.7246338957134,-12.8642531782837));
#40889=CARTESIAN_POINT('Ctrl Pts',(-19.4301618064496,16.7474743274646,-12.8684318563677));
#40890=CARTESIAN_POINT('Ctrl Pts',(-19.5124365775469,16.7707241575398,-12.8726854342531));
#40891=CARTESIAN_POINT('Ctrl Pts',(-19.5936389405811,16.7981265494107,-12.8769390121385));
#40892=CARTESIAN_POINT('Ctrl Pts',(-19.673322970079,16.8295566649861,-12.881192590024));
#40893=CARTESIAN_POINT('Ctrl Pts',(-19.7514621691743,16.8603774464402,-12.8853637040019));
#40894=CARTESIAN_POINT('Ctrl Pts',(-19.8281409334347,16.8950709981006,-12.8895348179799));
#40895=CARTESIAN_POINT('Ctrl Pts',(-19.9029545672469,16.933469490937,-12.8937059319578));
#40896=CARTESIAN_POINT('Ctrl Pts',(-19.9777430966217,16.9718550987884,-12.8978756462782));
#40897=CARTESIAN_POINT('Ctrl Pts',(-20.0506673295888,17.013942968857,-12.9020453605985));
#40898=CARTESIAN_POINT('Ctrl Pts',(-20.1213450915267,17.0595182787166,-12.9062150749189));
#40899=CARTESIAN_POINT('Ctrl Pts',(-20.1920203384466,17.1050919668111,-12.9103846408629));
#40900=CARTESIAN_POINT('Ctrl Pts',(-20.2604488871165,17.154152597935,-12.914554206807));
#40901=CARTESIAN_POINT('Ctrl Pts',(-20.3262767630686,17.2064415174927,-12.918723772751));
#40902=CARTESIAN_POINT('Ctrl Pts',(-20.3944190659318,17.2605688509569,-12.9230399354899));
#40903=CARTESIAN_POINT('Ctrl Pts',(-20.4597740011395,17.3181553818452,-12.9273560982289));
#40904=CARTESIAN_POINT('Ctrl Pts',(-20.5219870028021,17.3788694157318,-12.9316722609678));
#40905=CARTESIAN_POINT('Ctrl Pts',(-20.5821734224789,17.4376056963504,-12.9358478251595));
#40906=CARTESIAN_POINT('Ctrl Pts',(-20.6394191762099,17.4992684748645,-12.9400233893511));
#40907=CARTESIAN_POINT('Ctrl Pts',(-20.69344276075,17.5635219068696,-12.9441989535428));
#40908=CARTESIAN_POINT('Ctrl Pts',(-20.7501949481165,17.6310206269775,-12.9485854155554));
#40909=CARTESIAN_POINT('Ctrl Pts',(-20.8033905562328,17.7013781204553,-12.9529718775679));
#40910=CARTESIAN_POINT('Ctrl Pts',(-20.8527544426649,17.7741702913401,-12.9573583395805));
#40911=CARTESIAN_POINT('Ctrl Pts',(-20.902118329097,17.8469624622249,-12.961744801593));
#40912=CARTESIAN_POINT('Ctrl Pts',(-20.9476502584793,17.9221887747549,-12.9661312636056));
#40913=CARTESIAN_POINT('Ctrl Pts',(-20.9891316170534,17.9993971815128,-12.9705177256181));
#40914=CARTESIAN_POINT('Ctrl Pts',(-21.030861876244,18.0770688619123,-12.9749305077209));
#40915=CARTESIAN_POINT('Ctrl Pts',(-21.0686351706118,18.1570094498411,-12.9793432898236));
#40916=CARTESIAN_POINT('Ctrl Pts',(-21.1022126120114,18.2388019624017,-12.9837560719264));
#40917=CARTESIAN_POINT('Ctrl Pts',(-21.1356929152443,18.3203578525637,-12.9881560880307));
#40918=CARTESIAN_POINT('Ctrl Pts',(-21.1650014030465,18.4037546379829,-12.992556104135));
#40919=CARTESIAN_POINT('Ctrl Pts',(-21.1899457627446,18.4885524860192,-12.9969561202393));
#40920=CARTESIAN_POINT('Ctrl Pts',(-21.2148467487812,18.5732028861678,-13.0013484855235));
#40921=CARTESIAN_POINT('Ctrl Pts',(-21.2353985968836,18.6592491335648,-13.0057408508078));
#40922=CARTESIAN_POINT('Ctrl Pts',(-21.2514572537725,18.7462323425323,-13.010133216092));
#40923=CARTESIAN_POINT('Ctrl Pts',(-21.267478998332,18.8330156124333,-13.0145154851125));
#40924=CARTESIAN_POINT('Ctrl Pts',(-21.2790280568695,18.9207311752703,-13.018897754133));
#40925=CARTESIAN_POINT('Ctrl Pts',(-21.28601069243,19.0089073833049,-13.0232800231535));
#40926=CARTESIAN_POINT('Ctrl Pts',(-21.291327328341,19.0760454703582,-13.0266167186811));
#40927=CARTESIAN_POINT('Ctrl Pts',(-21.2939976088987,19.1434502453364,-13.0299534142087));
#40928=CARTESIAN_POINT('Ctrl Pts',(-21.293999998394,19.2109093211998,-13.0332901097364));
#40929=CARTESIAN_POINT('Ctrl Pts',(-21.293999998394,19.2109093219103,-13.0332901097715));
#40930=CARTESIAN_POINT('Ctrl Pts',(-21.2940031178915,19.2989781543512,-13.0376462156856));
#40931=CARTESIAN_POINT('Ctrl Pts',(-21.2894573285641,19.3869643923453,-13.0420023215996));
#40932=CARTESIAN_POINT('Ctrl Pts',(-21.2804139262415,19.4743934627951,-13.0463584275137));
#40933=CARTESIAN_POINT('Ctrl Pts',(-21.2713470661107,19.5620493167382,-13.0507258327921));
#40934=CARTESIAN_POINT('Ctrl Pts',(-21.2577593163574,19.6491447181139,-13.0550932380704));
#40935=CARTESIAN_POINT('Ctrl Pts',(-21.2397536148681,19.7352125728896,-13.0594606433488));
#40936=CARTESIAN_POINT('Ctrl Pts',(-21.2217244341811,19.8213926590148,-13.0638337436661));
#40937=CARTESIAN_POINT('Ctrl Pts',(-21.1992659159006,19.9065421429604,-13.0682068439834));
#40938=CARTESIAN_POINT('Ctrl Pts',(-21.1725309633218,19.9902090482796,-13.0725799443008));
#40939=CARTESIAN_POINT('Ctrl Pts',(-21.1457232584227,20.0741036316349,-13.0769649448896));
#40940=CARTESIAN_POINT('Ctrl Pts',(-21.1146159900528,20.1565071961892,-13.0813499454785));
#40941=CARTESIAN_POINT('Ctrl Pts',(-21.0794107185111,20.2369866283209,-13.0857349460674));
#40942=CARTESIAN_POINT('Ctrl Pts',(-21.0474072811092,20.3101466511123,-13.0897211414781));
#40943=CARTESIAN_POINT('Ctrl Pts',(-21.0120180507083,20.3817167133685,-13.0937073368888));
#40944=CARTESIAN_POINT('Ctrl Pts',(-20.9734262024017,20.4513911818442,-13.0976935322996));
#40945=CARTESIAN_POINT('Ctrl Pts',(-20.9329131921061,20.524534153289,-13.1018781666926));
#40946=CARTESIAN_POINT('Ctrl Pts',(-20.8887375841055,20.5958263313022,-13.1060628010856));
#40947=CARTESIAN_POINT('Ctrl Pts',(-20.8410930441,20.6648771968448,-13.1102474354787));
#40948=CARTESIAN_POINT('Ctrl Pts',(-20.7935163201999,20.7338297770273,-13.1144261135626));
#40949=CARTESIAN_POINT('Ctrl Pts',(-20.7424807309407,20.8005470061349,-13.1186047916466));
#40950=CARTESIAN_POINT('Ctrl Pts',(-20.6882255495784,20.8646633579344,-13.1227834697305));
#40951=CARTESIAN_POINT('Ctrl Pts',(-20.6329978830828,20.9299289492601,-13.127037047616));
#40952=CARTESIAN_POINT('Ctrl Pts',(-20.574434300428,20.992499082944,-13.1312906255014));
#40953=CARTESIAN_POINT('Ctrl Pts',(-20.51283306354,21.0520195360334,-13.1355442033868));
#40954=CARTESIAN_POINT('Ctrl Pts',(-20.4524260868341,21.1103860689951,-13.1397153173648));
#40955=CARTESIAN_POINT('Ctrl Pts',(-20.3890985326089,21.1658197797782,-13.1438864313427));
#40956=CARTESIAN_POINT('Ctrl Pts',(-20.3231707254821,21.2180217749867,-13.1480575453207));
#40957=CARTESIAN_POINT('Ctrl Pts',(-20.2572650410675,21.2702062533116,-13.1522272596411));
#40958=CARTESIAN_POINT('Ctrl Pts',(-20.1887611969919,21.319160884427,-13.1563969739614));
#40959=CARTESIAN_POINT('Ctrl Pts',(-20.1180129698813,21.3646267316321,-13.1605666882818));
#40960=CARTESIAN_POINT('Ctrl Pts',(-20.0472672602961,21.4100909609673,-13.1647362542259));
#40961=CARTESIAN_POINT('Ctrl Pts',(-19.9742777139359,21.4520664052354,-13.1689058201699));
#40962=CARTESIAN_POINT('Ctrl Pts',(-19.8994263305446,21.4903379451221,-13.1730753861139));
#40963=CARTESIAN_POINT('Ctrl Pts',(-19.8219432648524,21.5299550651381,-13.1773915488529));
#40964=CARTESIAN_POINT('Ctrl Pts',(-19.7424654713774,21.5656027360313,-13.1817077115918));
#40965=CARTESIAN_POINT('Ctrl Pts',(-19.6614416802126,21.5970955407955,-13.1860238743307));
#40966=CARTESIAN_POINT('Ctrl Pts',(-19.5830572305228,21.627562470757,-13.1901994385224));
#40967=CARTESIAN_POINT('Ctrl Pts',(-19.5032264199663,21.6541409631941,-13.1943750027141));
#40968=CARTESIAN_POINT('Ctrl Pts',(-19.4223715061057,21.6767138255649,-13.1985505669058));
#40969=CARTESIAN_POINT('Ctrl Pts',(-19.3374328027603,21.7004267895521,-13.2029370289183));
#40970=CARTESIAN_POINT('Ctrl Pts',(-19.2513643920955,21.7197187126534,-13.2073234909308));
#40971=CARTESIAN_POINT('Ctrl Pts',(-19.1646662302709,21.7345147311051,-13.2117099529434));
#40972=CARTESIAN_POINT('Ctrl Pts',(-19.0779680684463,21.7493107495567,-13.2160964149559));
#40973=CARTESIAN_POINT('Ctrl Pts',(-18.9906407405947,21.7596108709354,-13.2204828769685));
#40974=CARTESIAN_POINT('Ctrl Pts',(-18.9031862415114,21.7654032601927,-13.224869338981));
#40975=CARTESIAN_POINT('Ctrl Pts',(-18.8197759389833,21.7709277894665,-13.229052955917));
#40976=CARTESIAN_POINT('Ctrl Pts',(-18.7359395737635,21.7723728408953,-13.233236572853));
#40977=CARTESIAN_POINT('Ctrl Pts',(-18.6521100212236,21.7696899052789,-13.237420189789));
#40978=CARTESIAN_POINT('Ctrl Pts',(-18.5683906915354,21.7670104973064,-13.241598305918));
#40979=CARTESIAN_POINT('Ctrl Pts',(-18.4846786121261,21.7602138920958,-13.245776422047));
#40980=CARTESIAN_POINT('Ctrl Pts',(-18.4014104699563,21.7493034106476,-13.249954538176));
#40981=CARTESIAN_POINT('Ctrl Pts',(-18.3182268241359,21.7384040006107,-13.2541284145615));
#40982=CARTESIAN_POINT('Ctrl Pts',(-18.2354866744585,21.7233990640566,-13.2583022909471));
#40983=CARTESIAN_POINT('Ctrl Pts',(-18.153624027431,21.7043438853204,-13.2624761673326));
#40984=CARTESIAN_POINT('Ctrl Pts',(-18.071819888646,21.6853023255552,-13.2666470605973));
#40985=CARTESIAN_POINT('Ctrl Pts',(-17.9908924531492,21.6622163790631,-13.2708179538619));
#40986=CARTESIAN_POINT('Ctrl Pts',(-17.9112665890495,21.6351925943509,-13.2749888471266));
#40987=CARTESIAN_POINT('Ctrl Pts',(-17.8316596834536,21.6081752438612,-13.2791587473233));
#40988=CARTESIAN_POINT('Ctrl Pts',(-17.753354171139,21.5772220585794,-13.2833286475199));
#40989=CARTESIAN_POINT('Ctrl Pts',(-17.6767596812528,21.5424894184652,-13.2874985477166));
#40990=CARTESIAN_POINT('Ctrl Pts',(-17.6001752728601,21.5077613499186,-13.2916678990641));
#40991=CARTESIAN_POINT('Ctrl Pts',(-17.5253018556168,21.469255010947,-13.2958372504116));
#40992=CARTESIAN_POINT('Ctrl Pts',(-17.4525274999561,21.4271742331394,-13.3000066017591));
#40993=CARTESIAN_POINT('Ctrl Pts',(-17.3797189214394,21.3850736664325,-13.3041779137851));
#40994=CARTESIAN_POINT('Ctrl Pts',(-17.3090117699117,21.339395541617,-13.3083492258111));
#40995=CARTESIAN_POINT('Ctrl Pts',(-17.2407671572916,21.2903882940559,-13.312520537837));
#40996=CARTESIAN_POINT('Ctrl Pts',(-17.2183978647968,21.2743246457625,-13.3138878149775));
#40997=CARTESIAN_POINT('Ctrl Pts',(-17.1962929040477,21.2579036529085,-13.315255092118));
#40998=CARTESIAN_POINT('Ctrl Pts',(-17.1744642439897,21.2411350264762,-13.3166223692584));
#40999=CARTESIAN_POINT('',(-21.2943302428071,19.2116425108278,-12.9667098340901));
#41000=CARTESIAN_POINT('Ctrl Pts',(-21.2939999191096,19.2116435515775,-12.9667098902285));
#41001=CARTESIAN_POINT('Ctrl Pts',(-21.2939911726516,19.2464363059257,-12.9684506873211));
#41002=CARTESIAN_POINT('Ctrl Pts',(-21.2932731600888,19.281219269613,-12.9701914844137));
#41003=CARTESIAN_POINT('Ctrl Pts',(-21.2918468828523,19.3159729673895,-12.9719322815063));
#41004=CARTESIAN_POINT('Ctrl Pts',(-21.2884183105029,19.3995160291397,-12.9761169158993));
#41005=CARTESIAN_POINT('Ctrl Pts',(-21.2808860937369,19.4830464110296,-12.9803015502924));
#41006=CARTESIAN_POINT('Ctrl Pts',(-21.2692483017375,19.5661282142231,-12.9844861846854));
#41007=CARTESIAN_POINT('Ctrl Pts',(-21.2576270746945,19.6490917607532,-12.9886648627693));
#41008=CARTESIAN_POINT('Ctrl Pts',(-21.2419119432712,19.7316075451531,-12.9928435408533));
#41009=CARTESIAN_POINT('Ctrl Pts',(-21.2221529486456,19.8132415662722,-12.9970222189372));
#41010=CARTESIAN_POINT('Ctrl Pts',(-21.2020397882419,19.8963388185507,-13.0012757968227));
#41011=CARTESIAN_POINT('Ctrl Pts',(-21.1777363859676,19.9785219036746,-13.0055293747081));
#41012=CARTESIAN_POINT('Ctrl Pts',(-21.1493505801535,20.0593404829147,-13.0097829525936));
#41013=CARTESIAN_POINT('Ctrl Pts',(-21.1215150885756,20.1385922362917,-13.0139540665715));
#41014=CARTESIAN_POINT('Ctrl Pts',(-21.0897542310845,20.2165314648403,-13.0181251805494));
#41015=CARTESIAN_POINT('Ctrl Pts',(-21.0542203695085,20.292747399774,-13.0222962945274));
#41016=CARTESIAN_POINT('Ctrl Pts',(-21.018698431663,20.3689377597145,-13.0264660088478));
#41017=CARTESIAN_POINT('Ctrl Pts',(-20.9794061983923,20.4434055578918,-13.0306357231681));
#41018=CARTESIAN_POINT('Ctrl Pts',(-20.9365438451405,20.5157607482728,-13.0348054374885));
#41019=CARTESIAN_POINT('Ctrl Pts',(-20.8936830171152,20.5881133639457,-13.0389750034325));
#41020=CARTESIAN_POINT('Ctrl Pts',(-20.8472525568965,20.6583531259272,-13.0431445693766));
#41021=CARTESIAN_POINT('Ctrl Pts',(-20.7974975099507,20.7261165058923,-13.0473141353206));
#41022=CARTESIAN_POINT('Ctrl Pts',(-20.7459931369336,20.796262362702,-13.0516302980595));
#41023=CARTESIAN_POINT('Ctrl Pts',(-20.6909263546122,20.8637540331552,-13.0559464607985));
#41024=CARTESIAN_POINT('Ctrl Pts',(-20.6326151733211,20.928224628182,-13.0602626235374));
#41025=CARTESIAN_POINT('Ctrl Pts',(-20.5762034726275,20.9905951003567,-13.0644381877291));
#41026=CARTESIAN_POINT('Ctrl Pts',(-20.5167558657732,21.0501379976125,-13.0686137519207));
#41027=CARTESIAN_POINT('Ctrl Pts',(-20.4545972806998,21.1065592836016,-13.0727893161124));
#41028=CARTESIAN_POINT('Ctrl Pts',(-20.389299213262,21.1658302746175,-13.077175778125));
#41029=CARTESIAN_POINT('Ctrl Pts',(-20.321009559389,21.2216556522273,-13.0815622401375));
#41030=CARTESIAN_POINT('Ctrl Pts',(-20.2501416763133,21.2737443897259,-13.0859487021501));
#41031=CARTESIAN_POINT('Ctrl Pts',(-20.1792737932376,21.3258331272245,-13.0903351641626));
#41032=CARTESIAN_POINT('Ctrl Pts',(-20.1058282074104,21.3741849690991,-13.0947216261752));
#41033=CARTESIAN_POINT('Ctrl Pts',(-20.0302483510418,21.4185643167123,-13.0991080881878));
#41034=CARTESIAN_POINT('Ctrl Pts',(-19.9581460359011,21.4609017047557,-13.1032927225808));
#41035=CARTESIAN_POINT('Ctrl Pts',(-19.8838331576255,21.4997817138927,-13.1074773569739));
#41036=CARTESIAN_POINT('Ctrl Pts',(-19.8076751930389,21.5349667768393,-13.1116619913669));
#41037=CARTESIAN_POINT('Ctrl Pts',(-19.7316256298885,21.5701017582038,-13.1158406694508));
#41038=CARTESIAN_POINT('Ctrl Pts',(-19.6537366110357,21.6015520487104,-13.1200193475348));
#41039=CARTESIAN_POINT('Ctrl Pts',(-19.5744001491065,21.629124808479,-13.1241980256187));
#41040=CARTESIAN_POINT('Ctrl Pts',(-19.4936416381154,21.6571917901503,-13.1284516035042));
#41041=CARTESIAN_POINT('Ctrl Pts',(-19.4113836985809,21.6812406201864,-13.1327051813896));
#41042=CARTESIAN_POINT('Ctrl Pts',(-19.3280633649497,21.701118213745,-13.136958759275));
#41043=CARTESIAN_POINT('Ctrl Pts',(-19.2463583585722,21.7206104413645,-13.141129873253));
#41044=CARTESIAN_POINT('Ctrl Pts',(-19.1636322517455,21.7360916126581,-13.1453009872309));
#41045=CARTESIAN_POINT('Ctrl Pts',(-19.0803129065814,21.7474674984583,-13.1494721012089));
#41046=CARTESIAN_POINT('Ctrl Pts',(-18.9970215200282,21.7588395669701,-13.1536418155293));
#41047=CARTESIAN_POINT('Ctrl Pts',(-18.9131377459123,21.76610902368,-13.1578115298496));
#41048=CARTESIAN_POINT('Ctrl Pts',(-18.8290979023926,21.7692330599381,-13.16198124417));
#41049=CARTESIAN_POINT('Ctrl Pts',(-18.7450610493711,21.7723569850297,-13.166150810114));
#41050=CARTESIAN_POINT('Ctrl Pts',(-18.6608685977348,21.7713357667235,-13.1703203760581));
#41051=CARTESIAN_POINT('Ctrl Pts',(-18.5769588557388,21.7661786784898,-13.1744899420021));
#41052=CARTESIAN_POINT('Ctrl Pts',(-18.4900989507282,21.7608402733959,-13.178806104741));
#41053=CARTESIAN_POINT('Ctrl Pts',(-18.4035425318193,21.7510697851063,-13.18312226748));
#41054=CARTESIAN_POINT('Ctrl Pts',(-18.3177702276211,21.7369360198915,-13.1874384302189));
#41055=CARTESIAN_POINT('Ctrl Pts',(-18.2347919472105,21.7232626605919,-13.1916139944106));
#41056=CARTESIAN_POINT('Ctrl Pts',(-18.1525479314088,21.7055060719794,-13.1957895586022));
#41057=CARTESIAN_POINT('Ctrl Pts',(-18.0714612955845,21.6837803107335,-13.1999651227939));
#41058=CARTESIAN_POINT('Ctrl Pts',(-17.98627916655,21.6609572329353,-13.2043515848065));
#41059=CARTESIAN_POINT('Ctrl Pts',(-17.9023749641125,21.6337536591884,-13.208738046819));
#41060=CARTESIAN_POINT('Ctrl Pts',(-17.8202171381048,21.6023596302745,-13.2131245088315));
#41061=CARTESIAN_POINT('Ctrl Pts',(-17.7380593120971,21.5709656013606,-13.2175109708441));
#41062=CARTESIAN_POINT('Ctrl Pts',(-17.6576483623233,21.5353814216376,-13.2218974328566));
#41063=CARTESIAN_POINT('Ctrl Pts',(-17.579422411398,21.4958524223455,-13.2262838948691));
#41064=CARTESIAN_POINT('Ctrl Pts',(-17.5048157787013,21.4581523305451,-13.2304674063041));
#41065=CARTESIAN_POINT('Ctrl Pts',(-17.4319187998215,21.4167240952405,-13.2346509177391));
#41066=CARTESIAN_POINT('Ctrl Pts',(-17.361128739488,21.3717462835928,-13.238834429174));
#41067=CARTESIAN_POINT('Ctrl Pts',(-17.2970900087018,21.3310580576203,-13.2426189543074));
#41068=CARTESIAN_POINT('Ctrl Pts',(-17.2347755193382,21.2874657331385,-13.2464034794408));
#41069=CARTESIAN_POINT('Ctrl Pts',(-17.1744642439897,21.2411350264762,-13.2501880045741));
#41070=CARTESIAN_POINT('Ctrl Pts',(-17.1725834302249,21.2436206685575,-12.4500366781978));
#41071=CARTESIAN_POINT('Ctrl Pts',(-17.1023021618046,21.1904720651656,-12.4544341370588));
#41072=CARTESIAN_POINT('Ctrl Pts',(-16.3858468952195,20.5851355922428,-12.5012235314802));
#41073=CARTESIAN_POINT('Ctrl Pts',(-15.7591748512996,18.6509044920109,-12.590404861462));
#41074=CARTESIAN_POINT('Ctrl Pts',(-17.5947352542129,16.4064737508063,-12.7175806681434));
#41075=CARTESIAN_POINT('Ctrl Pts',(-20.4360629288883,16.7305239810473,-12.8430154491748));
#41076=CARTESIAN_POINT('Ctrl Pts',(-21.2952860172943,18.397872866616,-12.9260582946456));
#41077=CARTESIAN_POINT('Ctrl Pts',(-21.2980344808449,19.2116308398979,-12.9667092045559));
#41078=CARTESIAN_POINT('Origin',(-18.734,19.211,1.76670989022852));
#41079=CARTESIAN_POINT('',(-17.1744642439897,21.2411350264762,-11.6500725230732));
#41080=CARTESIAN_POINT('',(-17.1744642439897,21.2411350264762,-11.7167617806966));
#41081=CARTESIAN_POINT('',(-17.1744642439897,21.2411350264762,1.76670989022852));
#41082=CARTESIAN_POINT('',(-21.2939989766127,19.2087109517328,-12.2332901098107));
#41083=CARTESIAN_POINT('Ctrl Pts',(-17.1744642439897,21.2411350264762,-11.7167617806966));
#41084=CARTESIAN_POINT('Ctrl Pts',(-17.1079833326068,21.1900648478714,-11.7209383054901));
#41085=CARTESIAN_POINT('Ctrl Pts',(-17.0439255876479,21.1356580021043,-11.7251148302835));
#41086=CARTESIAN_POINT('Ctrl Pts',(-16.9826417696875,21.0781755003525,-11.7292913550769));
#41087=CARTESIAN_POINT('Ctrl Pts',(-16.9214168264467,21.0207482214358,-11.7334638675269));
#41088=CARTESIAN_POINT('Ctrl Pts',(-16.8629608482341,20.960251472191,-11.7376363799769));
#41089=CARTESIAN_POINT('Ctrl Pts',(-16.807591531515,20.8969864805358,-11.7418088924268));
#41090=CARTESIAN_POINT('Ctrl Pts',(-16.7522505048174,20.8337538130643,-11.7459792730017));
#41091=CARTESIAN_POINT('Ctrl Pts',(-16.6999933106994,20.7677560570195,-11.7501496535766));
#41092=CARTESIAN_POINT('Ctrl Pts',(-16.6510999429969,20.6993303909201,-11.7543200341515));
#41093=CARTESIAN_POINT('Ctrl Pts',(-16.6022168895844,20.6309191595426,-11.7584895349646));
#41094=CARTESIAN_POINT('Ctrl Pts',(-16.5566965201686,20.5600814098146,-11.7626590357778));
#41095=CARTESIAN_POINT('Ctrl Pts',(-16.5147769260435,20.4871853110027,-11.7668285365909));
#41096=CARTESIAN_POINT('Ctrl Pts',(-16.4728536003033,20.4142827230967,-11.7709984085663));
#41097=CARTESIAN_POINT('Ctrl Pts',(-16.4345319145091,20.3393218217299,-11.7751682805418));
#41098=CARTESIAN_POINT('Ctrl Pts',(-16.4000045262528,20.2626963100285,-11.7793381525172));
#41099=CARTESIAN_POINT('Ctrl Pts',(-16.3654407311331,20.185990001757,-11.7835124213488));
#41100=CARTESIAN_POINT('Ctrl Pts',(-16.3346794113464,20.1076159987801,-11.7876866901803));
#41101=CARTESIAN_POINT('Ctrl Pts',(-16.3078652590156,20.0279885057873,-11.7918609590119));
#41102=CARTESIAN_POINT('Ctrl Pts',(-16.2810362895517,19.948317011733,-11.7960375344873));
#41103=CARTESIAN_POINT('Ctrl Pts',(-16.2581589557103,19.86739109131,-11.8002141099626));
#41104=CARTESIAN_POINT('Ctrl Pts',(-16.2393275127547,19.785638304833,-11.8043906854379));
#41105=CARTESIAN_POINT('Ctrl Pts',(-16.2204635694863,19.7037444250189,-11.8085744690709));
#41106=CARTESIAN_POINT('Ctrl Pts',(-16.2056595438309,19.621021282185,-11.8127582527039));
#41107=CARTESIAN_POINT('Ctrl Pts',(-16.1949581671405,19.5379045288606,-11.8169420363368));
#41108=CARTESIAN_POINT('Ctrl Pts',(-16.1872903014398,19.4783488174401,-11.819939846053));
#41109=CARTESIAN_POINT('Ctrl Pts',(-16.1817277091854,19.4185911599263,-11.8229376557691));
#41110=CARTESIAN_POINT('Ctrl Pts',(-16.1782696504243,19.3587916785811,-11.8259354654852));
#41111=CARTESIAN_POINT('Ctrl Pts',(-16.1734425556468,19.2753177459375,-11.8301200998783));
#41112=CARTESIAN_POINT('Ctrl Pts',(-16.172700351485,19.1914517330296,-11.8343047342713));
#41113=CARTESIAN_POINT('Ctrl Pts',(-16.1760879473577,19.1076272233757,-11.8384893686644));
#41114=CARTESIAN_POINT('Ctrl Pts',(-16.1794707214069,19.0239220275358,-11.8426680467483));
#41115=CARTESIAN_POINT('Ctrl Pts',(-16.1869716010008,18.940258673335,-11.8468467248323));
#41116=CARTESIAN_POINT('Ctrl Pts',(-16.1985835897659,18.8570739812961,-11.8510254029162));
#41117=CARTESIAN_POINT('Ctrl Pts',(-16.2104037150842,18.772398263436,-11.8552789808016));
#41118=CARTESIAN_POINT('Ctrl Pts',(-16.2264838103268,18.6882190178967,-11.8595325586871));
#41119=CARTESIAN_POINT('Ctrl Pts',(-16.246760974914,18.604995023049,-11.8637861365725));
#41120=CARTESIAN_POINT('Ctrl Pts',(-16.2666450270981,18.5233844877397,-11.8679572505505));
#41121=CARTESIAN_POINT('Ctrl Pts',(-16.2905647501885,18.4426929623941,-11.8721283645284));
#41122=CARTESIAN_POINT('Ctrl Pts',(-16.3184090347916,18.3633442392081,-11.8762994785064));
#41123=CARTESIAN_POINT('Ctrl Pts',(-16.3462439759762,18.2840221422525,-11.8804691928267));
#41124=CARTESIAN_POINT('Ctrl Pts',(-16.3780007110433,18.2060423862984,-11.8846389071471));
#41125=CARTESIAN_POINT('Ctrl Pts',(-16.4135185064012,18.1298128571494,-11.8888086214675));
#41126=CARTESIAN_POINT('Ctrl Pts',(-16.4490350378836,18.0535860405741,-11.8929781874115));
#41127=CARTESIAN_POINT('Ctrl Pts',(-16.4883121684969,17.9791097436056,-11.8971477533556));
#41128=CARTESIAN_POINT('Ctrl Pts',(-16.5311418982014,17.9067698886546,-11.9013173192996));
#41129=CARTESIAN_POINT('Ctrl Pts',(-16.5754774683661,17.8318866536443,-11.9056334820385));
#41130=CARTESIAN_POINT('Ctrl Pts',(-16.6236198358012,17.7592933443554,-11.9099496447775));
#41131=CARTESIAN_POINT('Ctrl Pts',(-16.6752887227188,17.6893864233008,-11.9142658075164));
#41132=CARTESIAN_POINT('Ctrl Pts',(-16.7252745010797,17.6217567128467,-11.9184413717081));
#41133=CARTESIAN_POINT('Ctrl Pts',(-16.7785602395925,17.5566413947911,-11.9226169358997));
#41134=CARTESIAN_POINT('Ctrl Pts',(-16.8348515919039,17.4943651162737,-11.9267925000914));
#41135=CARTESIAN_POINT('Ctrl Pts',(-16.8939860866005,17.4289434109761,-11.931178962104));
#41136=CARTESIAN_POINT('Ctrl Pts',(-16.9564373882605,17.3666554945532,-11.9355654241165));
#41137=CARTESIAN_POINT('Ctrl Pts',(-17.0218228555023,17.3078317400031,-11.9399518861291));
#41138=CARTESIAN_POINT('Ctrl Pts',(-17.087208322744,17.249007985453,-11.9443383481416));
#41139=CARTESIAN_POINT('Ctrl Pts',(-17.1555274568811,17.1936486989612,-11.9487248101541));
#41140=CARTESIAN_POINT('Ctrl Pts',(-17.2263622218886,17.142032061628,-11.9531112721667));
#41141=CARTESIAN_POINT('Ctrl Pts',(-17.2939377743557,17.0927903822928,-11.9572959065597));
#41142=CARTESIAN_POINT('Ctrl Pts',(-17.3640540780912,17.0467712239068,-11.9614805409528));
#41143=CARTESIAN_POINT('Ctrl Pts',(-17.436370866589,17.0042470387189,-11.9656651753458));
#41144=CARTESIAN_POINT('Ctrl Pts',(-17.5085847210893,16.9617833814452,-11.9698438534298));
#41145=CARTESIAN_POINT('Ctrl Pts',(-17.5829924458181,16.9228050473159,-11.9740225315137));
#41146=CARTESIAN_POINT('Ctrl Pts',(-17.6592229568397,16.8875425961521,-11.9782012095977));
#41147=CARTESIAN_POINT('Ctrl Pts',(-17.7368198449855,16.8516480908938,-11.9824547874831));
#41148=CARTESIAN_POINT('Ctrl Pts',(-17.8163051194014,16.8196042772378,-11.9867083653685));
#41149=CARTESIAN_POINT('Ctrl Pts',(-17.8972589731898,16.7916065937817,-11.990961943254));
#41150=CARTESIAN_POINT('Ctrl Pts',(-17.9766433785541,16.7641517000524,-11.9951330572319));
#41151=CARTESIAN_POINT('Ctrl Pts',(-18.0574394740944,16.7405876095594,-11.9993041712099));
#41152=CARTESIAN_POINT('Ctrl Pts',(-18.1392307762333,16.721050287564,-12.0034752851878));
#41153=CARTESIAN_POINT('Ctrl Pts',(-18.2209946325108,16.7015195215058,-12.0076449995082));
#41154=CARTESIAN_POINT('Ctrl Pts',(-18.303752585082,16.6860129471901,-12.0118147138286));
#41155=CARTESIAN_POINT('Ctrl Pts',(-18.3870746644909,16.6746161939521,-12.0159844281489));
#41156=CARTESIAN_POINT('Ctrl Pts',(-18.4703937789426,16.6632198462596,-12.020153994093));
#41157=CARTESIAN_POINT('Ctrl Pts',(-18.554276524415,16.6559330903703,-12.024323560037));
#41158=CARTESIAN_POINT('Ctrl Pts',(-18.6382858147575,16.6527899236491,-12.0284931259811));
#41159=CARTESIAN_POINT('Ctrl Pts',(-18.7252487681118,16.6495362470634,-12.03280928872));
#41160=CARTESIAN_POINT('Ctrl Pts',(-18.8123468034838,16.6507229779045,-12.0371254514589));
#41161=CARTESIAN_POINT('Ctrl Pts',(-18.8990948495911,16.6563290445464,-12.0414416141978));
#41162=CARTESIAN_POINT('Ctrl Pts',(-18.9830170872208,16.6617524941571,-12.0456171783895));
#41163=CARTESIAN_POINT('Ctrl Pts',(-19.066611324596,16.6713116809416,-12.0497927425812));
#41164=CARTESIAN_POINT('Ctrl Pts',(-19.1494452607506,16.6849348315374,-12.0539683067729));
#41165=CARTESIAN_POINT('Ctrl Pts',(-19.2364629421014,16.6992460550838,-12.0583547687854));
#41166=CARTESIAN_POINT('Ctrl Pts',(-19.3226409276423,16.7180424488712,-12.0627412307979));
#41167=CARTESIAN_POINT('Ctrl Pts',(-19.4074943094423,16.7411810966897,-12.0671276928105));
#41168=CARTESIAN_POINT('Ctrl Pts',(-19.4923476912424,16.7643197445083,-12.071514154823));
#41169=CARTESIAN_POINT('Ctrl Pts',(-19.5758759419184,16.7918003927741,-12.0759006168356));
#41170=CARTESIAN_POINT('Ctrl Pts',(-19.6576188802165,16.8234221134992,-12.0802870788481));
#41171=CARTESIAN_POINT('Ctrl Pts',(-19.7356007047514,16.8535888719792,-12.0844717132412));
#41172=CARTESIAN_POINT('Ctrl Pts',(-19.8122481596155,16.8876362896631,-12.0886563476342));
#41173=CARTESIAN_POINT('Ctrl Pts',(-19.8871479757777,16.9254257295026,-12.0928409820273));
#41174=CARTESIAN_POINT('Ctrl Pts',(-19.9619411813225,16.9631613807519,-12.0970196601112));
#41175=CARTESIAN_POINT('Ctrl Pts',(-20.0349912820117,17.0046282689895,-12.1011983381951));
#41176=CARTESIAN_POINT('Ctrl Pts',(-20.1059035528266,17.0496391690091,-12.1053770162791));
#41177=CARTESIAN_POINT('Ctrl Pts',(-20.1780868751321,17.0954568570628,-12.1096305941645));
#41178=CARTESIAN_POINT('Ctrl Pts',(-20.2480545228571,17.1449466854561,-12.11388417205));
#41179=CARTESIAN_POINT('Ctrl Pts',(-20.3154149295587,17.1978614502303,-12.1181377499354));
#41180=CARTESIAN_POINT('Ctrl Pts',(-20.3814694233333,17.2497503590347,-12.1223088639133));
#41181=CARTESIAN_POINT('Ctrl Pts',(-20.4450164884365,17.3049322938692,-12.1264799778913));
#41182=CARTESIAN_POINT('Ctrl Pts',(-20.5057163649394,17.3631306533724,-12.1306510918693));
#41183=CARTESIAN_POINT('Ctrl Pts',(-20.5663958730124,17.4213094838539,-12.1348208061896));
#41184=CARTESIAN_POINT('Ctrl Pts',(-20.6242297581414,17.4825024106647,-12.13899052051));
#41185=CARTESIAN_POINT('Ctrl Pts',(-20.678913285295,17.5463942470714,-12.1431602348304));
#41186=CARTESIAN_POINT('Ctrl Pts',(-20.733594866574,17.6102838099324,-12.1473298007744));
#41187=CARTESIAN_POINT('Ctrl Pts',(-20.7851260142849,17.6768717413838,-12.1514993667185));
#41188=CARTESIAN_POINT('Ctrl Pts',(-20.8332415555807,17.7458089232721,-12.1556689326625));
#41189=CARTESIAN_POINT('Ctrl Pts',(-20.8830487799516,17.8171698514324,-12.1599850954014));
#41190=CARTESIAN_POINT('Ctrl Pts',(-20.9291954417205,17.8910478705134,-12.1643012581404));
#41191=CARTESIAN_POINT('Ctrl Pts',(-20.971436698905,17.9670237066595,-12.1686174208793));
#41192=CARTESIAN_POINT('Ctrl Pts',(-21.0123019515797,18.0405246379345,-12.172792985071));
#41193=CARTESIAN_POINT('Ctrl Pts',(-21.0495121634691,18.1159883689943,-12.1769685492626));
#41194=CARTESIAN_POINT('Ctrl Pts',(-21.082893688299,18.1930125535797,-12.1811441134543));
#41195=CARTESIAN_POINT('Ctrl Pts',(-21.117961234591,18.2739270466209,-12.1855305754669));
#41196=CARTESIAN_POINT('Ctrl Pts',(-21.1488029510882,18.3565632259543,-12.1899170374794));
#41197=CARTESIAN_POINT('Ctrl Pts',(-21.1752765362398,18.4404360029143,-12.1943034994919));
#41198=CARTESIAN_POINT('Ctrl Pts',(-21.2017501213915,18.5243087798743,-12.1986899615045));
#41199=CARTESIAN_POINT('Ctrl Pts',(-21.2238555029592,18.6094175737551,-12.203076423517));
#41200=CARTESIAN_POINT('Ctrl Pts',(-21.2415125421985,18.6952666864385,-12.2074628855296));
#41201=CARTESIAN_POINT('Ctrl Pts',(-21.2654843862328,18.8118185902907,-12.2134181072291));
#41202=CARTESIAN_POINT('Ctrl Pts',(-21.2813366135111,18.9300931627089,-12.2193733289286));
#41203=CARTESIAN_POINT('Ctrl Pts',(-21.2888788651003,19.0491544419404,-12.2253285506281));
#41204=CARTESIAN_POINT('Ctrl Pts',(-21.2922399536336,19.1022122716411,-12.2279824036759));
#41205=CARTESIAN_POINT('Ctrl Pts',(-21.2939513313562,19.1554260264004,-12.2306362567237));
#41206=CARTESIAN_POINT('Ctrl Pts',(-21.293998976612,19.2087109509454,-12.2332901097715));
#41207=CARTESIAN_POINT('Ctrl Pts',(-21.2939989766127,19.2087109517328,-12.2332901098107));
#41208=CARTESIAN_POINT('Ctrl Pts',(-21.2940747905548,19.2934988599292,-12.2375129674107));
#41209=CARTESIAN_POINT('Ctrl Pts',(-21.2899336304853,19.3784221563149,-12.2417358250107));
#41210=CARTESIAN_POINT('Ctrl Pts',(-21.2815646644668,19.4630203967141,-12.2459586826108));
#41211=CARTESIAN_POINT('Ctrl Pts',(-21.2734134565487,19.5454174151129,-12.2500716626647));
#41212=CARTESIAN_POINT('Ctrl Pts',(-21.2612518149666,19.6275055813485,-12.2541846427187));
#41213=CARTESIAN_POINT('Ctrl Pts',(-21.2451224198776,19.7088596111236,-12.2582976227727));
#41214=CARTESIAN_POINT('Ctrl Pts',(-21.2290007459442,19.7901746966529,-12.2624086339395));
#41215=CARTESIAN_POINT('Ctrl Pts',(-21.20891517906,19.8707558783839,-12.2665196451063));
#41216=CARTESIAN_POINT('Ctrl Pts',(-21.18495989447,19.9501857653523,-12.2706306562731));
#41217=CARTESIAN_POINT('Ctrl Pts',(-21.1610084101081,20.0296030516903,-12.2747410152757));
#41218=CARTESIAN_POINT('Ctrl Pts',(-21.1331885645307,20.1078689519367,-12.2788513742782));
#41219=CARTESIAN_POINT('Ctrl Pts',(-21.1016446063279,20.184580514455,-12.2829617332808));
#41220=CARTESIAN_POINT('Ctrl Pts',(-21.0685960771618,20.2649510340633,-12.2872681465249));
#41221=CARTESIAN_POINT('Ctrl Pts',(-21.0314595036716,20.3436147061448,-12.2915745597691));
#41222=CARTESIAN_POINT('Ctrl Pts',(-20.9904568914614,20.4201328698601,-12.2958809730133));
#41223=CARTESIAN_POINT('Ctrl Pts',(-20.9512718262788,20.4932591677037,-12.2999964933322));
#41224=CARTESIAN_POINT('Ctrl Pts',(-20.9085564982548,20.5644257408166,-12.304112013651));
#41225=CARTESIAN_POINT('Ctrl Pts',(-20.8625501361321,20.6332778624348,-12.3082275339699));
#41226=CARTESIAN_POINT('Ctrl Pts',(-20.8165130556112,20.70217595654,-12.3123458022172));
#41227=CARTESIAN_POINT('Ctrl Pts',(-20.7671808550876,20.768756147345,-12.3164640704645));
#41228=CARTESIAN_POINT('Ctrl Pts',(-20.7148334041511,20.8326963417974,-12.3205823387118));
#41229=CARTESIAN_POINT('Ctrl Pts',(-20.662405465351,20.8967348487665,-12.3247069390843));
#41230=CARTESIAN_POINT('Ctrl Pts',(-20.6069533520093,20.9581249187391,-12.3288315394568));
#41231=CARTESIAN_POINT('Ctrl Pts',(-20.5487934990216,21.0165815007661,-12.3329561398293));
#41232=CARTESIAN_POINT('Ctrl Pts',(-20.5408850965646,21.0245302515484,-12.3335169906232));
#41233=CARTESIAN_POINT('Ctrl Pts',(-20.5329266770598,21.0324248251517,-12.3340778414171));
#41234=CARTESIAN_POINT('Ctrl Pts',(-20.5249190804941,21.040264564551,-12.334638692211));
#41235=CARTESIAN_POINT('Ctrl Pts',(-20.4651725946906,21.0987586301398,-12.338823326604));
#41236=CARTESIAN_POINT('Ctrl Pts',(-20.4024461555817,21.154431359773,-12.3430079609971));
#41237=CARTESIAN_POINT('Ctrl Pts',(-20.3370370650428,21.2069639696395,-12.3471925953901));
#41238=CARTESIAN_POINT('Ctrl Pts',(-20.2717210762482,21.2594218058381,-12.3513712734741));
#41239=CARTESIAN_POINT('Ctrl Pts',(-20.2037303762194,21.3087481146436,-12.355549951558));
#41240=CARTESIAN_POINT('Ctrl Pts',(-20.1333988170805,21.35466110912,-12.3597286296419));
#41241=CARTESIAN_POINT('Ctrl Pts',(-20.0618066152904,21.4013970610254,-12.3639822075274));
#41242=CARTESIAN_POINT('Ctrl Pts',(-19.9877891536758,21.4445957903898,-12.3682357854128));
#41243=CARTESIAN_POINT('Ctrl Pts',(-19.9117335730787,21.484003218397,-12.3724893632982));
#41244=CARTESIAN_POINT('Ctrl Pts',(-19.8371524783218,21.522646656515,-12.3766604772762));
#41245=CARTESIAN_POINT('Ctrl Pts',(-19.7606120124672,21.5576442636059,-12.3808315912541));
#41246=CARTESIAN_POINT('Ctrl Pts',(-19.6825046263017,21.5888012898231,-12.3850027052321));
#41247=CARTESIAN_POINT('Ctrl Pts',(-19.604423449824,21.6199478609992,-12.3891724195525));
#41248=CARTESIAN_POINT('Ctrl Pts',(-19.5247768242091,21.647256240463,-12.3933421338728));
#41249=CARTESIAN_POINT('Ctrl Pts',(-19.4439778217472,21.6705795357392,-12.3975118481932));
#41250=CARTESIAN_POINT('Ctrl Pts',(-19.3631816944606,21.6939020010724,-12.4016814141372));
#41251=CARTESIAN_POINT('Ctrl Pts',(-19.2812337140822,21.713239537401,-12.4058509800813));
#41252=CARTESIAN_POINT('Ctrl Pts',(-19.1985614595125,21.7284953128726,-12.4100205460253));
#41253=CARTESIAN_POINT('Ctrl Pts',(-19.1129825504592,21.7442874625898,-12.4143367087642));
#41254=CARTESIAN_POINT('Ctrl Pts',(-19.0266280073017,21.7557053858608,-12.4186528715032));
#41255=CARTESIAN_POINT('Ctrl Pts',(-18.9399808515256,21.762699803818,-12.4229690342421));
#41256=CARTESIAN_POINT('Ctrl Pts',(-18.8561562177353,21.7694663793458,-12.4271445984338));
#41257=CARTESIAN_POINT('Ctrl Pts',(-18.7720582145671,21.7720932477196,-12.4313201626255));
#41258=CARTESIAN_POINT('Ctrl Pts',(-18.688124977799,21.7705889283903,-12.4354957268171));
#41259=CARTESIAN_POINT('Ctrl Pts',(-18.599952472774,21.7690086294678,-12.4398821888297));
#41260=CARTESIAN_POINT('Ctrl Pts',(-18.5119623987478,21.7628688832023,-12.4442686508422));
#41261=CARTESIAN_POINT('Ctrl Pts',(-18.4246552312347,21.7522409988109,-12.4486551128548));
#41262=CARTESIAN_POINT('Ctrl Pts',(-18.3373480637217,21.7416131144196,-12.4530415748673));
#41263=CARTESIAN_POINT('Ctrl Pts',(-18.2507243612258,21.7264972665758,-12.4574280368799));
#41264=CARTESIAN_POINT('Ctrl Pts',(-18.1652685194105,21.7070257416514,-12.4618144988924));
#41265=CARTESIAN_POINT('Ctrl Pts',(-18.0837368018496,21.6884483473282,-12.4659995349801));
#41266=CARTESIAN_POINT('Ctrl Pts',(-18.0029645350277,21.6658373731168,-12.4701845710677));
#41267=CARTESIAN_POINT('Ctrl Pts',(-17.9233808127673,21.6392702759969,-12.4743696071554));
#41268=CARTESIAN_POINT('Ctrl Pts',(-17.8439306160917,21.6127477531578,-12.4785476215887));
#41269=CARTESIAN_POINT('Ctrl Pts',(-17.7656654318222,21.5822824489659,-12.482725636022));
#41270=CARTESIAN_POINT('Ctrl Pts',(-17.6890027068815,21.5480024940883,-12.4869036504553));
#41271=CARTESIAN_POINT('Ctrl Pts',(-17.6124142566805,21.5137557513712,-12.4910776170161));
#41272=CARTESIAN_POINT('Ctrl Pts',(-17.5374256011855,21.4757018817769,-12.4952515835769));
#41273=CARTESIAN_POINT('Ctrl Pts',(-17.4644368058601,21.4340180602247,-12.4994255501377));
#41274=CARTESIAN_POINT('Ctrl Pts',(-17.3915013099496,21.3923646779103,-12.5035964686968));
#41275=CARTESIAN_POINT('Ctrl Pts',(-17.3205631705258,21.3470868385412,-12.5077673872559));
#41276=CARTESIAN_POINT('Ctrl Pts',(-17.251999007923,21.2984082158224,-12.511938305815));
#41277=CARTESIAN_POINT('Ctrl Pts',(-17.2258011156292,21.2798084507762,-12.5135319849474));
#41278=CARTESIAN_POINT('Ctrl Pts',(-17.1999495451948,21.2607126594728,-12.5151256640799));
#41279=CARTESIAN_POINT('Ctrl Pts',(-17.1744642439897,21.2411350264762,-12.5167193432124));
#41280=CARTESIAN_POINT('',(-21.2939992159918,19.2130035272629,-12.1667098902285));
#41281=CARTESIAN_POINT('Ctrl Pts',(-21.2916489709697,19.2130199896839,-12.1667107986323));
#41282=CARTESIAN_POINT('Ctrl Pts',(-21.2937097175741,19.4962014444643,-12.1807663462274));
#41283=CARTESIAN_POINT('Ctrl Pts',(-21.1196060444512,20.6310006101477,-12.2372138293831));
#41284=CARTESIAN_POINT('Ctrl Pts',(-19.5298543885185,22.0831545624874,-12.3316557892382));
#41285=CARTESIAN_POINT('Ctrl Pts',(-17.7798204959642,21.7028298248134,-12.4120422014983));
#41286=CARTESIAN_POINT('Ctrl Pts',(-17.1725834302249,21.2436206685575,-12.4500366781978));
#41287=CARTESIAN_POINT('Ctrl Pts',(-17.1744642439897,21.2411350264762,-11.6500725230732));
#41288=CARTESIAN_POINT('Ctrl Pts',(-17.1077138936498,21.189857866719,-11.6542476640414));
#41289=CARTESIAN_POINT('Ctrl Pts',(-17.0435214358735,21.1353053413385,-11.6584228050097));
#41290=CARTESIAN_POINT('Ctrl Pts',(-16.9822123288039,21.0777726040001,-11.6625979459779));
#41291=CARTESIAN_POINT('Ctrl Pts',(-16.9208932902774,21.0202305469385,-11.6667737632768));
#41292=CARTESIAN_POINT('Ctrl Pts',(-16.8624588433937,20.9597076574843,-11.6709495805758));
#41293=CARTESIAN_POINT('Ctrl Pts',(-16.807196255566,20.8965347313049,-11.6751253978747));
#41294=CARTESIAN_POINT('Ctrl Pts',(-16.7518333577028,20.8332471366179,-11.6793087949197));
#41295=CARTESIAN_POINT('Ctrl Pts',(-16.6996541106652,20.7673002542451,-11.6834921919647));
#41296=CARTESIAN_POINT('Ctrl Pts',(-16.6509045356354,20.6990568827647,-11.6876755890097));
#41297=CARTESIAN_POINT('Ctrl Pts',(-16.6023552598585,20.6310939054482,-11.6918417975705));
#41298=CARTESIAN_POINT('Ctrl Pts',(-16.5572076916088,20.5608537004042,-11.6960080061312));
#41299=CARTESIAN_POINT('Ctrl Pts',(-16.5156592733602,20.4887184433712,-11.7001742146919));
#41300=CARTESIAN_POINT('Ctrl Pts',(-16.4739270995035,20.4162641547462,-11.704358849085));
#41301=CARTESIAN_POINT('Ctrl Pts',(-16.4356706929266,20.341628329944,-11.708543483478));
#41302=CARTESIAN_POINT('Ctrl Pts',(-16.4011245523601,20.2651784221843,-11.712728117871));
#41303=CARTESIAN_POINT('Ctrl Pts',(-16.3666275839488,20.1888373314056,-11.716906795955));
#41304=CARTESIAN_POINT('Ctrl Pts',(-16.3358305794285,20.1106877022102,-11.7210854740389));
#41305=CARTESIAN_POINT('Ctrl Pts',(-16.3089230895031,20.0311231481764,-11.7252641521229));
#41306=CARTESIAN_POINT('Ctrl Pts',(-16.2815333021588,19.9501324566934,-11.7295177300083));
#41307=CARTESIAN_POINT('Ctrl Pts',(-16.258174080664,19.8676760341798,-11.7337713078938));
#41308=CARTESIAN_POINT('Ctrl Pts',(-16.2389948450999,19.7841921815777,-11.7380248857792));
#41309=CARTESIAN_POINT('Ctrl Pts',(-16.2201874364424,19.7023268263637,-11.7421959997571));
#41310=CARTESIAN_POINT('Ctrl Pts',(-16.2053994934178,19.6194739920342,-11.7463671137351));
#41311=CARTESIAN_POINT('Ctrl Pts',(-16.194721659298,19.5360623147052,-11.7505382277131));
#41312=CARTESIAN_POINT('Ctrl Pts',(-16.1840474082286,19.4526786269702,-11.7547079420334));
#41313=CARTESIAN_POINT('Ctrl Pts',(-16.1774805853424,19.3687369245932,-11.7588776563538));
#41314=CARTESIAN_POINT('Ctrl Pts',(-16.1750603443919,19.2846738688843,-11.7630473706742));
#41315=CARTESIAN_POINT('Ctrl Pts',(-16.172640189564,19.2006138044998,-11.7672169366182));
#41316=CARTESIAN_POINT('Ctrl Pts',(-16.1743663356855,19.1164328552362,-11.7713865025623));
#41317=CARTESIAN_POINT('Ctrl Pts',(-16.1802258395509,19.0325692363342,-11.7755560685063));
#41318=CARTESIAN_POINT('Ctrl Pts',(-16.1862913563437,18.9457570760485,-11.7798722312452));
#41319=CARTESIAN_POINT('Ctrl Pts',(-16.1967862597981,18.8592855021225,-11.7841883939841));
#41320=CARTESIAN_POINT('Ctrl Pts',(-16.2116377216372,18.7736345501845,-11.7885045567231));
#41321=CARTESIAN_POINT('Ctrl Pts',(-16.226005398669,18.6907736689971,-11.7926801209147));
#41322=CARTESIAN_POINT('Ctrl Pts',(-16.2444500136974,18.6086812165377,-11.7968556851064));
#41323=CARTESIAN_POINT('Ctrl Pts',(-16.2668539711945,18.527779338318,-11.8010312492981));
#41324=CARTESIAN_POINT('Ctrl Pts',(-16.2903894993245,18.4427912985553,-11.8054177113106));
#41325=CARTESIAN_POINT('Ctrl Pts',(-16.3182946694534,18.3591178195347,-11.8098041733232));
#41326=CARTESIAN_POINT('Ctrl Pts',(-16.3503755250187,18.2772257434101,-11.8141906353357));
#41327=CARTESIAN_POINT('Ctrl Pts',(-16.382456380584,18.1953336672856,-11.8185770973483));
#41328=CARTESIAN_POINT('Ctrl Pts',(-16.4187126130535,18.1152234912951,-11.8229635593608));
#41329=CARTESIAN_POINT('Ctrl Pts',(-16.4588952312817,18.0373312684769,-11.8273500213734));
#41330=CARTESIAN_POINT('Ctrl Pts',(-16.4972289876803,17.9630229822945,-11.8315346557664));
#41331=CARTESIAN_POINT('Ctrl Pts',(-16.5392784376737,17.8904564421858,-11.8357192901595));
#41332=CARTESIAN_POINT('Ctrl Pts',(-16.5848615409703,17.8200277199314,-11.8399039245525));
#41333=CARTESIAN_POINT('Ctrl Pts',(-16.6303797623612,17.749699244246,-11.8440826026365));
#41334=CARTESIAN_POINT('Ctrl Pts',(-16.6794213986321,17.6815029251176,-11.8482612807204));
#41335=CARTESIAN_POINT('Ctrl Pts',(-16.7317580832552,17.6158112002556,-11.8524399588043));
#41336=CARTESIAN_POINT('Ctrl Pts',(-16.7850328653365,17.5489419984372,-11.8566935366898));
#41337=CARTESIAN_POINT('Ctrl Pts',(-16.8417217641062,17.4846684922401,-11.8609471145752));
#41338=CARTESIAN_POINT('Ctrl Pts',(-16.9015371160905,17.4233535642935,-11.8652006924606));
#41339=CARTESIAN_POINT('Ctrl Pts',(-16.9601928307565,17.3632273458715,-11.8693718064386));
#41340=CARTESIAN_POINT('Ctrl Pts',(-17.0218545195986,17.3059463582363,-11.8735429204166));
#41341=CARTESIAN_POINT('Ctrl Pts',(-17.0862108309601,17.2518188306349,-11.8777140343945));
#41342=CARTESIAN_POINT('Ctrl Pts',(-17.15054554694,17.1977094660481,-11.8818837487149));
#41343=CARTESIAN_POINT('Ctrl Pts',(-17.2175727378981,17.1467517558066,-11.8860534630352));
#41344=CARTESIAN_POINT('Ctrl Pts',(-17.2869464339594,17.0992149785054,-11.8902231773556));
#41345=CARTESIAN_POINT('Ctrl Pts',(-17.3563176614068,17.0516798927667,-11.8943927432997));
#41346=CARTESIAN_POINT('Ctrl Pts',(-17.4280348479702,17.0075657572679,-11.8985623092437));
#41347=CARTESIAN_POINT('Ctrl Pts',(-17.5017225180694,16.9670988864198,-11.9027318751878));
#41348=CARTESIAN_POINT('Ctrl Pts',(-17.5780009557457,16.9252092503139,-11.9070480379267));
#41349=CARTESIAN_POINT('Ctrl Pts',(-17.6563905571825,16.8872283803615,-11.9113642006656));
#41350=CARTESIAN_POINT('Ctrl Pts',(-17.7364482678186,16.8533548736882,-11.9156803634045));
#41351=CARTESIAN_POINT('Ctrl Pts',(-17.8138981069513,16.8205847929319,-11.9198559275962));
#41352=CARTESIAN_POINT('Ctrl Pts',(-17.8929085883425,16.7916587077374,-11.9240314917879));
#41353=CARTESIAN_POINT('Ctrl Pts',(-17.9730611021941,16.7667062382345,-11.9282070559796));
#41354=CARTESIAN_POINT('Ctrl Pts',(-18.0572619289758,16.7404934788158,-11.9325935179921));
#41355=CARTESIAN_POINT('Ctrl Pts',(-18.1427226225442,16.7186664436046,-11.9369799800047));
#41356=CARTESIAN_POINT('Ctrl Pts',(-18.2289456575188,16.7013147386294,-11.9413664420172));
#41357=CARTESIAN_POINT('Ctrl Pts',(-18.3151686924934,16.6839630336542,-11.9457529040297));
#41358=CARTESIAN_POINT('Ctrl Pts',(-18.4021534837731,16.6710866686339,-11.9501393660423));
#41359=CARTESIAN_POINT('Ctrl Pts',(-18.4893986055749,16.662712308658,-11.9545258280548));
#41360=CARTESIAN_POINT('Ctrl Pts',(-18.5726294499944,16.6547232653983,-11.9587104624479));
#41361=CARTESIAN_POINT('Ctrl Pts',(-18.6564069960725,16.6508013065455,-11.9628950968409));
#41362=CARTESIAN_POINT('Ctrl Pts',(-18.740299675164,16.6510077511655,-11.967079731234));
#41363=CARTESIAN_POINT('Ctrl Pts',(-18.8240729434104,16.6512139019371,-11.9712584093179));
#41364=CARTESIAN_POINT('Ctrl Pts',(-18.907960563061,16.655536782935,-11.9754370874018));
#41365=CARTESIAN_POINT('Ctrl Pts',(-18.9915257624718,16.6639859675174,-11.9796157654858));
#41366=CARTESIAN_POINT('Ctrl Pts',(-19.076588808025,16.6725865976611,-11.9838693433712));
#41367=CARTESIAN_POINT('Ctrl Pts',(-19.1613172809479,16.6854629604527,-11.9881229212567));
#41368=CARTESIAN_POINT('Ctrl Pts',(-19.2452503475945,16.702569597919,-11.9923764991421));
#41369=CARTESIAN_POINT('Ctrl Pts',(-19.3275562079622,16.7193445898371,-11.99654761312));
#41370=CARTESIAN_POINT('Ctrl Pts',(-19.4090967563144,16.7401871997923,-12.000718727098));
#41371=CARTESIAN_POINT('Ctrl Pts',(-19.4894442918863,16.7650024689595,-12.004889841076));
#41372=CARTESIAN_POINT('Ctrl Pts',(-19.5697648660668,16.7898094111234,-12.0090595553963));
#41373=CARTESIAN_POINT('Ctrl Pts',(-19.6488927833418,16.818586229372,-12.0132292697167));
#41374=CARTESIAN_POINT('Ctrl Pts',(-19.7264143560957,16.8511877731872,-12.0173989840371));
#41375=CARTESIAN_POINT('Ctrl Pts',(-19.8039331702993,16.8837881568995,-12.0215685499811));
#41376=CARTESIAN_POINT('Ctrl Pts',(-19.8798453299031,16.9202128164537,-12.0257381159252));
#41377=CARTESIAN_POINT('Ctrl Pts',(-19.9537573024926,16.9602685360053,-12.0299076818692));
#41378=CARTESIAN_POINT('Ctrl Pts',(-20.0302679288583,17.0017325652423,-12.0342238446081));
#41379=CARTESIAN_POINT('Ctrl Pts',(-20.1046346343667,17.0470874900863,-12.038540007347));
#41380=CARTESIAN_POINT('Ctrl Pts',(-20.1764506132331,17.0960682686234,-12.042856170086));
#41381=CARTESIAN_POINT('Ctrl Pts',(-20.2459271941416,17.1434535034516,-12.0470317342777));
#41382=CARTESIAN_POINT('Ctrl Pts',(-20.3130163291627,17.1942316733327,-12.0512072984693));
#41383=CARTESIAN_POINT('Ctrl Pts',(-20.377382442736,17.2481209545907,-12.055382862661));
#41384=CARTESIAN_POINT('Ctrl Pts',(-20.44499953569,17.3047320553354,-12.0597693246736));
#41385=CARTESIAN_POINT('Ctrl Pts',(-20.5096108706378,17.3647764140011,-12.0641557866861));
#41386=CARTESIAN_POINT('Ctrl Pts',(-20.5708718020377,17.4278841925218,-12.0685422486987));
#41387=CARTESIAN_POINT('Ctrl Pts',(-20.6321327334376,17.4909919710424,-12.0729287107112));
#41388=CARTESIAN_POINT('Ctrl Pts',(-20.6900429364134,17.5571626827011,-12.0773151727237));
#41389=CARTESIAN_POINT('Ctrl Pts',(-20.7443085775788,17.625989141074,-12.0817016347363));
#41390=CARTESIAN_POINT('Ctrl Pts',(-20.796026764239,17.6915845997261,-12.0858821780095));
#41391=CARTESIAN_POINT('Ctrl Pts',(-20.8446312405901,17.7598411080022,-12.0900627212828));
#41392=CARTESIAN_POINT('Ctrl Pts',(-20.8898359348525,17.8304307616065,-12.0942432645561));
#41393=CARTESIAN_POINT('Ctrl Pts',(-20.934977871844,17.9009224162288,-12.0984180040186));
#41394=CARTESIAN_POINT('Ctrl Pts',(-20.9767291512529,17.9737404018926,-12.1025927434812));
#41395=CARTESIAN_POINT('Ctrl Pts',(-21.0148441174676,18.0485241457073,-12.1067674829438));
#41396=CARTESIAN_POINT('Ctrl Pts',(-21.0529176328928,18.1232265607022,-12.1109376822936));
#41397=CARTESIAN_POINT('Ctrl Pts',(-21.087362480976,18.199890080528,-12.1151078816434));
#41398=CARTESIAN_POINT('Ctrl Pts',(-21.1179772351417,18.2781267276172,-12.1192780809931));
#41399=CARTESIAN_POINT('Ctrl Pts',(-21.1485693987601,18.3563056440885,-12.1234452031637));
#41400=CARTESIAN_POINT('Ctrl Pts',(-21.1753369141585,18.436054955007,-12.1276123253342));
#41401=CARTESIAN_POINT('Ctrl Pts',(-21.198125670353,18.5169649283305,-12.1317794475048));
#41402=CARTESIAN_POINT('Ctrl Pts',(-21.2209040463211,18.5978380473459,-12.1359446715607));
#41403=CARTESIAN_POINT('Ctrl Pts',(-21.2397071410263,18.6798703351908,-12.1401098956166));
#41404=CARTESIAN_POINT('Ctrl Pts',(-21.2544305326007,18.7626363860277,-12.1442751196726));
#41405=CARTESIAN_POINT('Ctrl Pts',(-21.2691564647158,18.8454167182569,-12.1484410624434));
#41406=CARTESIAN_POINT('Ctrl Pts',(-21.279801198365,18.9289306143289,-12.1526070052143));
#41407=CARTESIAN_POINT('Ctrl Pts',(-21.2863115236392,19.0127428783158,-12.1567729479852));
#41408=CARTESIAN_POINT('Ctrl Pts',(-21.2914878410454,19.0793814658917,-12.1600852620663));
#41409=CARTESIAN_POINT('Ctrl Pts',(-21.2940514917317,19.1462084026767,-12.1633975761474));
#41410=CARTESIAN_POINT('Ctrl Pts',(-21.2939992159918,19.2130035272629,-12.1667098902285));
#41411=CARTESIAN_POINT('Origin',(-18.734,19.211,1.76670989022852));
#41412=CARTESIAN_POINT('',(-17.1757181329867,21.2395346319231,-10.8502164826864));
#41413=CARTESIAN_POINT('',(-17.173194974388,21.2428171613069,-10.9165936635695));
#41414=CARTESIAN_POINT('',(-17.1744642439897,21.2411350264762,1.76670989022852));
#41415=CARTESIAN_POINT('',(-21.2940197026037,19.2123010442705,-11.4332901032639));
#41416=CARTESIAN_POINT('Ctrl Pts',(-17.173194974388,21.2428171613069,-10.9165936635695));
#41417=CARTESIAN_POINT('Ctrl Pts',(-17.0711420934188,21.1659200956527,-10.9229640486181));
#41418=CARTESIAN_POINT('Ctrl Pts',(-16.3366272634488,20.5183600625041,-10.9717263692271));
#41419=CARTESIAN_POINT('Ctrl Pts',(-15.788288410751,18.513809214,-11.0628806253966));
#41420=CARTESIAN_POINT('Ctrl Pts',(-17.7257693047706,16.3567465732145,-11.1900564320781));
#41421=CARTESIAN_POINT('Ctrl Pts',(-20.5048168878155,16.8048334715693,-11.3135258905415));
#41422=CARTESIAN_POINT('Ctrl Pts',(-21.2925957841654,18.43736680388,-11.3946034134446));
#41423=CARTESIAN_POINT('Ctrl Pts',(-21.297413587737,19.2122806855485,-11.4332890007871));
#41424=CARTESIAN_POINT('Ctrl Pts',(-21.2939996693303,19.212301164443,-11.4332901097715));
#41425=CARTESIAN_POINT('Ctrl Pts',(-21.293961988618,19.2864367677247,-11.436996088328));
#41426=CARTESIAN_POINT('Ctrl Pts',(-21.2907042434478,19.3604881810636,-11.4407020668845));
#41427=CARTESIAN_POINT('Ctrl Pts',(-21.2842464642989,19.4342553948533,-11.444408045441));
#41428=CARTESIAN_POINT('Ctrl Pts',(-21.2769546129518,19.5175502156942,-11.4485926798341));
#41429=CARTESIAN_POINT('Ctrl Pts',(-21.2655641024497,19.6006424250678,-11.4527773142271));
#41430=CARTESIAN_POINT('Ctrl Pts',(-21.250093180474,19.6830965019697,-11.4569619486202));
#41431=CARTESIAN_POINT('Ctrl Pts',(-21.2346442794409,19.7654332156989,-11.4611406267041));
#41432=CARTESIAN_POINT('Ctrl Pts',(-21.2151265874821,19.8471331528555,-11.465319304788));
#41433=CARTESIAN_POINT('Ctrl Pts',(-21.1916101807318,19.9277650937117,-11.469497982872));
#41434=CARTESIAN_POINT('Ctrl Pts',(-21.1676722592913,20.0098423041587,-11.4737515607574));
#41435=CARTESIAN_POINT('Ctrl Pts',(-21.1395909011584,20.0908123737399,-11.4780051386429));
#41436=CARTESIAN_POINT('Ctrl Pts',(-21.107494673889,20.170230437914,-11.4822587165283));
#41437=CARTESIAN_POINT('Ctrl Pts',(-21.0760206946157,20.2481088279425,-11.4864298305062));
#41438=CARTESIAN_POINT('Ctrl Pts',(-21.0406863094725,20.3244944066984,-11.4906009444842));
#41439=CARTESIAN_POINT('Ctrl Pts',(-21.0016627302193,20.3989838980282,-11.4947720584621));
#41440=CARTESIAN_POINT('Ctrl Pts',(-20.962652245705,20.4734483936899,-11.4989417727825));
#41441=CARTESIAN_POINT('Ctrl Pts',(-20.9199552389621,20.5460176583684,-11.5031114871029));
#41442=CARTESIAN_POINT('Ctrl Pts',(-20.873789724926,20.6163113295996,-11.5072812014233));
#41443=CARTESIAN_POINT('Ctrl Pts',(-20.827625853657,20.6866024994803,-11.5114507673673));
#41444=CARTESIAN_POINT('Ctrl Pts',(-20.7779939737414,20.7546178528605,-11.5156203333114));
#41445=CARTESIAN_POINT('Ctrl Pts',(-20.7251556946207,20.8200055934581,-11.5197898992554));
#41446=CARTESIAN_POINT('Ctrl Pts',(-20.6704596867893,20.8876922863505,-11.5241060619943));
#41447=CARTESIAN_POINT('Ctrl Pts',(-20.6123279420986,20.9525627446113,-11.5284222247332));
#41448=CARTESIAN_POINT('Ctrl Pts',(-20.5510951122121,21.0142651921375,-11.5327383874721));
#41449=CARTESIAN_POINT('Ctrl Pts',(-20.4918569353186,21.0739576889255,-11.5369139516638));
#41450=CARTESIAN_POINT('Ctrl Pts',(-20.4297169860235,21.1306851185865,-11.5410895158555));
#41451=CARTESIAN_POINT('Ctrl Pts',(-20.3650134540522,21.1841687998498,-11.5452650800472));
#41452=CARTESIAN_POINT('Ctrl Pts',(-20.2970419004992,21.2403538147082,-11.5496515420597));
#41453=CARTESIAN_POINT('Ctrl Pts',(-20.2262414538862,21.2929584378006,-11.5540380040723));
#41454=CARTESIAN_POINT('Ctrl Pts',(-20.1530384991425,21.3417110873958,-11.5584244660848));
#41455=CARTESIAN_POINT('Ctrl Pts',(-20.0798355443987,21.390463736991,-11.5628109280973));
#41456=CARTESIAN_POINT('Ctrl Pts',(-20.0042306192381,21.4353641822177,-11.5671973901099));
#41457=CARTESIAN_POINT('Ctrl Pts',(-19.9266775857363,21.4761976020829,-11.5715838521224));
#41458=CARTESIAN_POINT('Ctrl Pts',(-19.852692882267,21.5151522157705,-11.5757684865155));
#41459=CARTESIAN_POINT('Ctrl Pts',(-19.7766600165144,21.5505508359911,-11.5799531209085));
#41460=CARTESIAN_POINT('Ctrl Pts',(-19.6989550698443,21.5821730668978,-11.5841377553015));
#41461=CARTESIAN_POINT('Ctrl Pts',(-19.6213607265478,21.6137502874729,-11.5883164333855));
#41462=CARTESIAN_POINT('Ctrl Pts',(-19.5420994522195,21.6415616236984,-11.5924951114694));
#41463=CARTESIAN_POINT('Ctrl Pts',(-19.4615717652906,21.6654325874531,-11.5966737895534));
#41464=CARTESIAN_POINT('Ctrl Pts',(-19.3796006774477,21.6897314210775,-11.6009273674388));
#41465=CARTESIAN_POINT('Ctrl Pts',(-19.2963177561689,21.7099470058045,-11.6051809453242));
#41466=CARTESIAN_POINT('Ctrl Pts',(-19.2121666533117,21.7259466498637,-11.6094345232097));
#41467=CARTESIAN_POINT('Ctrl Pts',(-19.1296469837908,21.7416361096021,-11.6136056371876));
#41468=CARTESIAN_POINT('Ctrl Pts',(-19.0462929678286,21.7532715484977,-11.6177767511656));
#41469=CARTESIAN_POINT('Ctrl Pts',(-18.9625363705288,21.760778642813,-11.6219478651435));
#41470=CARTESIAN_POINT('Ctrl Pts',(-18.878807878564,21.7682832180503,-11.6261175794639));
#41471=CARTESIAN_POINT('Ctrl Pts',(-18.7946775313674,21.7716621589129,-11.6302872937843));
#41472=CARTESIAN_POINT('Ctrl Pts',(-18.7105831609272,21.7708928984721,-11.6344570081046));
#41473=CARTESIAN_POINT('Ctrl Pts',(-18.6264917829255,21.7701236654048,-11.6386265740487));
#41474=CARTESIAN_POINT('Ctrl Pts',(-18.5424368391406,21.7652065295826,-11.6427961399927));
#41475=CARTESIAN_POINT('Ctrl Pts',(-18.4588557388016,21.75617104249,-11.6469657059368));
#41476=CARTESIAN_POINT('Ctrl Pts',(-18.372336030083,21.7468178788176,-11.6512818686757));
#41477=CARTESIAN_POINT('Ctrl Pts',(-18.2863246298128,21.7330514297719,-11.6555980314146));
#41478=CARTESIAN_POINT('Ctrl Pts',(-18.2012984666221,21.7149626747092,-11.6599141941535));
#41479=CARTESIAN_POINT('Ctrl Pts',(-18.1190420217543,21.6974631589401,-11.6640897583452));
#41480=CARTESIAN_POINT('Ctrl Pts',(-18.0377080547437,21.6759187771978,-11.6682653225369));
#41481=CARTESIAN_POINT('Ctrl Pts',(-17.957713948121,21.6504630486355,-11.6724408867286));
#41482=CARTESIAN_POINT('Ctrl Pts',(-17.8736795293404,21.6237216117387,-11.6768273487411));
#41483=CARTESIAN_POINT('Ctrl Pts',(-17.7911244272666,21.592663525305,-11.6812138107537));
#41484=CARTESIAN_POINT('Ctrl Pts',(-17.710507793232,21.5575003095429,-11.6856002727662));
#41485=CARTESIAN_POINT('Ctrl Pts',(-17.6298911591974,21.5223370937809,-11.6899867347788));
#41486=CARTESIAN_POINT('Ctrl Pts',(-17.5512134783825,21.4830690758564,-11.6943731967913));
#41487=CARTESIAN_POINT('Ctrl Pts',(-17.4749010481796,21.4399616034209,-11.6987596588039));
#41488=CARTESIAN_POINT('Ctrl Pts',(-17.4021059540594,21.3988410087172,-11.7029439432541));
#41489=CARTESIAN_POINT('Ctrl Pts',(-17.3311919413494,21.3540740524414,-11.7071282277043));
#41490=CARTESIAN_POINT('Ctrl Pts',(-17.2625477971258,21.3058576120244,-11.7113125121546));
#41491=CARTESIAN_POINT('Ctrl Pts',(-17.2327489645208,21.2849265675333,-11.7131289350019));
#41492=CARTESIAN_POINT('Ctrl Pts',(-17.2033776234909,21.263346085628,-11.7149453578493));
#41493=CARTESIAN_POINT('Ctrl Pts',(-17.1744642439897,21.2411350264762,-11.7167617806966));
#41494=CARTESIAN_POINT('',(-21.2939995125392,19.2094201902091,-11.3667098902285));
#41495=CARTESIAN_POINT('Ctrl Pts',(-21.2939995125392,19.2094201902091,-11.3667098902285));
#41496=CARTESIAN_POINT('Ctrl Pts',(-21.2940518853803,19.2942876523606,-11.3709134538372));
#41497=CARTESIAN_POINT('Ctrl Pts',(-21.2898797137862,19.3791700299233,-11.3751170174459));
#41498=CARTESIAN_POINT('Ctrl Pts',(-21.2815050782104,19.4636220031829,-11.3793205810546));
#41499=CARTESIAN_POINT('Ctrl Pts',(-21.2731292177987,19.5480863280015,-11.3835247594572));
#41500=CARTESIAN_POINT('Ctrl Pts',(-21.2605497166712,19.6321196761629,-11.3877289378599));
#41501=CARTESIAN_POINT('Ctrl Pts',(-21.2438404672875,19.7152824890537,-11.3919331162626));
#41502=CARTESIAN_POINT('Ctrl Pts',(-21.2271240709727,19.7984808725961,-11.3961390928892));
#41503=CARTESIAN_POINT('Ctrl Pts',(-21.2062745049673,19.880807540606,-11.4003450695159));
#41504=CARTESIAN_POINT('Ctrl Pts',(-21.1814163656275,19.9618349574033,-11.4045510461425));
#41505=CARTESIAN_POINT('Ctrl Pts',(-21.1565238219895,20.0429745182095,-11.408762843948));
#41506=CARTESIAN_POINT('Ctrl Pts',(-21.1276117659035,20.1228108093803,-11.4129746417534));
#41507=CARTESIAN_POINT('Ctrl Pts',(-21.0948539828414,20.2009335693377,-11.4171864395589));
#41508=CARTESIAN_POINT('Ctrl Pts',(-21.0620694457195,20.2791201340097,-11.4214016772397));
#41509=CARTESIAN_POINT('Ctrl Pts',(-21.0254331231615,20.3555899771933,-11.4256169149205));
#41510=CARTESIAN_POINT('Ctrl Pts',(-20.9851650013542,20.4299569872141,-11.4298321526013));
#41511=CARTESIAN_POINT('Ctrl Pts',(-20.9448260993909,20.5044547137502,-11.4340547994973));
#41512=CARTESIAN_POINT('Ctrl Pts',(-20.9008428915854,20.5768418481601,-11.4382774463933));
#41513=CARTESIAN_POINT('Ctrl Pts',(-20.8534787082554,20.6467611240217,-11.4425000932893));
#41514=CARTESIAN_POINT('Ctrl Pts',(-20.8410561777284,20.6650993339886,-11.4436075959693));
#41515=CARTESIAN_POINT('Ctrl Pts',(-20.8284012848672,20.6832679625288,-11.4447150986492));
#41516=CARTESIAN_POINT('Ctrl Pts',(-20.8155192213964,20.7012609606902,-11.4458226013291));
#41517=CARTESIAN_POINT('Ctrl Pts',(-20.7668450946151,20.7692464566218,-11.4500072357222));
#41518=CARTESIAN_POINT('Ctrl Pts',(-20.7147461245074,20.8349713096213,-11.4541918701152));
#41519=CARTESIAN_POINT('Ctrl Pts',(-20.6594597008472,20.8980699275411,-11.4583765045082));
#41520=CARTESIAN_POINT('Ctrl Pts',(-20.6042519705679,20.9610787323882,-11.4625551825922));
#41521=CARTESIAN_POINT('Ctrl Pts',(-20.5458660991118,21.0214683841929,-11.4667338606761));
#41522=CARTESIAN_POINT('Ctrl Pts',(-20.4845818988862,21.0789033741851,-11.4709125387601));
#41523=CARTESIAN_POINT('Ctrl Pts',(-20.4221992234157,21.1373678450951,-11.4751661166455));
#41524=CARTESIAN_POINT('Ctrl Pts',(-20.356813572753,21.1927702956727,-11.4794196945309));
#41525=CARTESIAN_POINT('Ctrl Pts',(-20.2887620518457,21.2447932446885,-11.4836732724164));
#41526=CARTESIAN_POINT('Ctrl Pts',(-20.2220298424627,21.2958076273232,-11.4878443863943));
#41527=CARTESIAN_POINT('Ctrl Pts',(-20.1527345889112,21.3435720832561,-11.4920155003723));
#41528=CARTESIAN_POINT('Ctrl Pts',(-20.0812289339452,21.3878266351598,-11.4961866143502));
#41529=CARTESIAN_POINT('Ctrl Pts',(-20.0097472733922,21.4320663370212,-11.5003563286706));
#41530=CARTESIAN_POINT('Ctrl Pts',(-19.9360570753464,21.4727982320515,-11.504526042991));
#41531=CARTESIAN_POINT('Ctrl Pts',(-19.8605396057917,21.5098058892787,-11.5086957573114));
#41532=CARTESIAN_POINT('Ctrl Pts',(-19.7850248234728,21.5468122296147,-11.5128653232554));
#41533=CARTESIAN_POINT('Ctrl Pts',(-19.7076833123971,21.5800943939658,-11.5170348891994));
#41534=CARTESIAN_POINT('Ctrl Pts',(-19.6289193227218,21.6094827299397,-11.5212044551435));
#41535=CARTESIAN_POINT('Ctrl Pts',(-19.5473860883354,21.639904323552,-11.5255206178824));
#41536=CARTESIAN_POINT('Ctrl Pts',(-19.464328979673,21.6661529958307,-11.5298367806213));
#41537=CARTESIAN_POINT('Ctrl Pts',(-19.3802151086564,21.6880962906888,-11.5341529433602));
#41538=CARTESIAN_POINT('Ctrl Pts',(-19.2988412381409,21.7093247850249,-11.5383285075519));
#41539=CARTESIAN_POINT('Ctrl Pts',(-19.2164788667994,21.7265240396989,-11.5425040717436));
#41540=CARTESIAN_POINT('Ctrl Pts',(-19.1335609462711,21.7396263168398,-11.5466796359353));
#41541=CARTESIAN_POINT('Ctrl Pts',(-19.0464550386955,21.7533903588514,-11.5510660979478));
#41542=CARTESIAN_POINT('Ctrl Pts',(-18.9587365661206,21.7626326086006,-11.5554525599603));
#41543=CARTESIAN_POINT('Ctrl Pts',(-18.8709107816373,21.7673363311332,-11.5598390219729));
#41544=CARTESIAN_POINT('Ctrl Pts',(-18.783084997154,21.7720400536657,-11.5642254839854));
#41545=CARTESIAN_POINT('Ctrl Pts',(-18.6951524811213,21.7722053239559,-11.568611945998));
#41546=CARTESIAN_POINT('Ctrl Pts',(-18.6076132463771,21.7678782506229,-11.5729984080105));
#41547=CARTESIAN_POINT('Ctrl Pts',(-18.5241126314324,21.76375080668,-11.5771825007382));
#41548=CARTESIAN_POINT('Ctrl Pts',(-18.440659044576,21.7555210317039,-11.5813665934658));
#41549=CARTESIAN_POINT('Ctrl Pts',(-18.3576882161332,21.7431906407936,-11.5855506861935));
#41550=CARTESIAN_POINT('Ctrl Pts',(-18.2748290034154,21.7308768372256,-11.5897291503099));
#41551=CARTESIAN_POINT('Ctrl Pts',(-18.1924517105385,21.7144734377133,-11.5939076144262));
#41552=CARTESIAN_POINT('Ctrl Pts',(-18.1109898384596,21.6940340993666,-11.5980860785426));
#41553=CARTESIAN_POINT('Ctrl Pts',(-18.0265307131236,21.6728427297706,-11.6024182822535));
#41554=CARTESIAN_POINT('Ctrl Pts',(-17.9430561814231,21.6473126765418,-11.6067504859644));
#41555=CARTESIAN_POINT('Ctrl Pts',(-17.8610409295545,21.6175623742855,-11.6110826896752));
#41556=CARTESIAN_POINT('Ctrl Pts',(-17.7820790900159,21.5889196701608,-11.6152536062606));
#41557=CARTESIAN_POINT('Ctrl Pts',(-17.7044702726561,21.5563655566265,-11.6194245228459));
#41558=CARTESIAN_POINT('Ctrl Pts',(-17.6286235702152,21.5200567226632,-11.6235954394312));
#41559=CARTESIAN_POINT('Ctrl Pts',(-17.5528073927267,21.4837625014041,-11.6277646774065));
#41560=CARTESIAN_POINT('Ctrl Pts',(-17.4787523341875,21.4437167634057,-11.6319339153819));
#41561=CARTESIAN_POINT('Ctrl Pts',(-17.4068461738869,21.4001237337879,-11.6361031533573));
#41562=CARTESIAN_POINT('Ctrl Pts',(-17.3349387846982,21.356529959158,-11.6402724625856));
#41563=CARTESIAN_POINT('Ctrl Pts',(-17.2651807609245,21.309389009247,-11.6444417718139));
#41564=CARTESIAN_POINT('Ctrl Pts',(-17.1979329485559,21.2589497097018,-11.6486110810422));
#41565=CARTESIAN_POINT('Ctrl Pts',(-17.1900756294251,21.2530563183884,-11.6490982283859));
#41566=CARTESIAN_POINT('Ctrl Pts',(-17.1822525452959,21.2471179459407,-11.6495853757296));
#41567=CARTESIAN_POINT('Ctrl Pts',(-17.1744642439897,21.2411350264762,-11.6500725230732));
#41568=CARTESIAN_POINT('Ctrl Pts',(-17.1757181329864,21.2395346319229,-10.8502164826864));
#41569=CARTESIAN_POINT('Ctrl Pts',(-16.7160809592132,20.8801557260842,-10.8791841133254));
#41570=CARTESIAN_POINT('Ctrl Pts',(-15.8690423976421,19.6129801926267,-10.9505436795248));
#41571=CARTESIAN_POINT('Ctrl Pts',(-16.5533150821545,17.1114988848558,-11.0642951812848));
#41572=CARTESIAN_POINT('Ctrl Pts',(-19.3189847985123,16.2409689515226,-11.1914709879662));
#41573=CARTESIAN_POINT('Ctrl Pts',(-21.0857646400936,17.7107520667789,-11.2922755723032));
#41574=CARTESIAN_POINT('Ctrl Pts',(-21.2926072565653,18.8863578111491,-11.3506882210795));
#41575=CARTESIAN_POINT('Ctrl Pts',(-21.2907952889915,19.209402892007,-11.3667089342955));
#41576=CARTESIAN_POINT('Origin',(-18.734,19.211,1.76670989022852));
#41577=CARTESIAN_POINT('',(-17.1744642439897,21.2411350264762,-10.0501312698105));
#41578=CARTESIAN_POINT('',(-17.1744642439897,21.2411350264762,-10.1166694888401));
#41579=CARTESIAN_POINT('',(-17.1744642439897,21.2411350264762,1.76670989022852));
#41580=CARTESIAN_POINT('',(-21.2939995125392,19.2125798097912,-10.6332901097715));
#41581=CARTESIAN_POINT('Ctrl Pts',(-17.1744642439897,21.2411350264762,-10.1166694888401));
#41582=CARTESIAN_POINT('Ctrl Pts',(-17.107774487029,21.1899044141359,-10.1208396489562));
#41583=CARTESIAN_POINT('Ctrl Pts',(-17.0436266170067,21.1353956546449,-10.1250098090722));
#41584=CARTESIAN_POINT('Ctrl Pts',(-16.9823480872221,21.0778999910176,-10.1291799691882));
#41585=CARTESIAN_POINT('Ctrl Pts',(-16.9210022641563,21.0203411882798,-10.1333547087835));
#41586=CARTESIAN_POINT('Ctrl Pts',(-16.8625324062092,20.9597892501365,-10.1375294483788));
#41587=CARTESIAN_POINT('Ctrl Pts',(-16.8072292781277,20.8965724800006,-10.1417041879741));
#41588=CARTESIAN_POINT('Ctrl Pts',(-16.7518918721062,20.8333165268977,-10.1458815151531));
#41589=CARTESIAN_POINT('Ctrl Pts',(-16.6997253880396,20.7673928147154,-10.1500588423321));
#41590=CARTESIAN_POINT('Ctrl Pts',(-16.6509789452328,20.6991610414859,-10.1542361695111));
#41591=CARTESIAN_POINT('Ctrl Pts',(-16.6021520613839,20.6308166726572,-10.1584203900864));
#41592=CARTESIAN_POINT('Ctrl Pts',(-16.5567567322681,20.5601570268823,-10.1626046106618));
#41593=CARTESIAN_POINT('Ctrl Pts',(-16.5149973626627,20.4875685627846,-10.1667888312371));
#41594=CARTESIAN_POINT('Ctrl Pts',(-16.4954988829386,20.4536752183978,-10.1687425470336));
#41595=CARTESIAN_POINT('Ctrl Pts',(-16.4767924376755,20.4193616721457,-10.1706962628301));
#41596=CARTESIAN_POINT('Ctrl Pts',(-16.4588952312818,20.3846687315233,-10.1726499786266));
#41597=CARTESIAN_POINT('Ctrl Pts',(-16.4205614748832,20.310360445341,-10.1768346130197));
#41598=CARTESIAN_POINT('Ctrl Pts',(-16.3858007370466,20.2340338438633,-10.1810192474127));
#41599=CARTESIAN_POINT('Ctrl Pts',(-16.3548302568732,20.1560668406995,-10.1852038818058));
#41600=CARTESIAN_POINT('Ctrl Pts',(-16.3239038593449,20.0782108139144,-10.1893825598897));
#41601=CARTESIAN_POINT('Ctrl Pts',(-16.2967571717625,19.9987194471875,-10.1935612379736));
#41602=CARTESIAN_POINT('Ctrl Pts',(-16.2735613224931,19.9179947059407,-10.1977399160576));
#41603=CARTESIAN_POINT('Ctrl Pts',(-16.2499497042962,19.8358230317228,-10.201993493943));
#41604=CARTESIAN_POINT('Ctrl Pts',(-16.2304321761497,19.7523737600805,-10.2062470718285));
#41605=CARTESIAN_POINT('Ctrl Pts',(-16.2151377103691,19.6680916383785,-10.2105006497139));
#41606=CARTESIAN_POINT('Ctrl Pts',(-16.2001397576524,19.5854434900687,-10.2146717636918));
#41607=CARTESIAN_POINT('Ctrl Pts',(-16.189202669843,19.5019949698567,-10.2188428776698));
#41608=CARTESIAN_POINT('Ctrl Pts',(-16.1823971528001,19.4181784500405,-10.2230139916478));
#41609=CARTESIAN_POINT('Ctrl Pts',(-16.1755939194142,19.3343900556671,-10.2271837059681));
#41610=CARTESIAN_POINT('Ctrl Pts',(-16.1729195406043,19.2502343650766,-10.2313534202885));
#41611=CARTESIAN_POINT('Ctrl Pts',(-16.1743929164357,19.1661493838669,-10.2355231346089));
#41612=CARTESIAN_POINT('Ctrl Pts',(-16.1758662398381,19.0820673947618,-10.2396927005529));
#41613=CARTESIAN_POINT('Ctrl Pts',(-16.1814870155133,18.9980565699821,-10.243862266497));
#41614=CARTESIAN_POINT('Ctrl Pts',(-16.1912220304803,18.9145540559813,-10.248031832441));
#41615=CARTESIAN_POINT('Ctrl Pts',(-16.2012993165641,18.8281156965995,-10.2523479951799));
#41616=CARTESIAN_POINT('Ctrl Pts',(-16.2157854771196,18.742222581345,-10.2566641579188));
#41617=CARTESIAN_POINT('Ctrl Pts',(-16.2345855425418,18.6573508603375,-10.2609803206578));
#41618=CARTESIAN_POINT('Ctrl Pts',(-16.2527731978103,18.575243826715,-10.2651558848494));
#41619=CARTESIAN_POINT('Ctrl Pts',(-16.2749978531258,18.4940931072454,-10.2693314490411));
#41620=CARTESIAN_POINT('Ctrl Pts',(-16.3011224991716,18.4143149518393,-10.2735070132328));
#41621=CARTESIAN_POINT('Ctrl Pts',(-16.3285666389837,18.3305073914581,-10.2778934752454));
#41622=CARTESIAN_POINT('Ctrl Pts',(-16.3603148903335,18.2482152402676,-10.2822799372579));
#41623=CARTESIAN_POINT('Ctrl Pts',(-16.396151895843,18.1678958623946,-10.2866663992705));
#41624=CARTESIAN_POINT('Ctrl Pts',(-16.4319889013525,18.0875764845217,-10.291052861283));
#41625=CARTESIAN_POINT('Ctrl Pts',(-16.4719143298048,18.0092303623903,-10.2954393232955));
#41626=CARTESIAN_POINT('Ctrl Pts',(-16.5156592733601,17.9332815566289,-10.2998257853081));
#41627=CARTESIAN_POINT('Ctrl Pts',(-16.5573914472168,17.8608272680038,-10.3040104197011));
#41628=CARTESIAN_POINT('Ctrl Pts',(-16.6027547120117,17.7902848467578,-10.3081950540942));
#41629=CARTESIAN_POINT('Ctrl Pts',(-16.6515488896105,17.7220415140652,-10.3123796884872));
#41630=CARTESIAN_POINT('Ctrl Pts',(-16.7002736147368,17.65389531731,-10.3165583665712));
#41631=CARTESIAN_POINT('Ctrl Pts',(-16.7524192872619,17.5880420799734,-10.3207370446551));
#41632=CARTESIAN_POINT('Ctrl Pts',(-16.8077405464177,17.5248432701896,-10.324915722739));
#41633=CARTESIAN_POINT('Ctrl Pts',(-16.8640533993853,17.4605116671605,-10.3291693006245));
#41634=CARTESIAN_POINT('Ctrl Pts',(-16.9236565628965,17.3989310067058,-10.3334228785099));
#41635=CARTESIAN_POINT('Ctrl Pts',(-16.9862458850684,17.3404504674456,-10.3376764563954));
#41636=CARTESIAN_POINT('Ctrl Pts',(-17.047621791097,17.2831036875543,-10.3418475703733));
#41637=CARTESIAN_POINT('Ctrl Pts',(-17.1118687523877,17.2287382262738,-10.3460186843513));
#41638=CARTESIAN_POINT('Ctrl Pts',(-17.1786614840028,17.1776475709667,-10.3501897983292));
#41639=CARTESIAN_POINT('Ctrl Pts',(-17.2454318026718,17.1265740596224,-10.3543595126496));
#41640=CARTESIAN_POINT('Ctrl Pts',(-17.3147458300055,17.0787734510952,-10.35852922697));
#41641=CARTESIAN_POINT('Ctrl Pts',(-17.3862455028589,17.0344987214716,-10.3626989412903));
#41642=CARTESIAN_POINT('Ctrl Pts',(-17.4577426314469,16.990225567333,-10.3668685072344));
#41643=CARTESIAN_POINT('Ctrl Pts',(-17.5314248593519,16.9494782841069,-10.3710380731784));
#41644=CARTESIAN_POINT('Ctrl Pts',(-17.6069066380297,16.9124655640164,-10.3752076391224));
#41645=CARTESIAN_POINT('Ctrl Pts',(-17.6850422629292,16.8741515223475,-10.3795238018614));
#41646=CARTESIAN_POINT('Ctrl Pts',(-17.7651058639349,16.8398397766947,-10.3838399646003));
#41647=CARTESIAN_POINT('Ctrl Pts',(-17.8466456689027,16.8097082036781,-10.3881561273392));
#41648=CARTESIAN_POINT('Ctrl Pts',(-17.9255293233002,16.7805581634832,-10.3923316915309));
#41649=CARTESIAN_POINT('Ctrl Pts',(-18.0057940203927,16.7553202361718,-10.3965072557226));
#41650=CARTESIAN_POINT('Ctrl Pts',(-18.087015599334,16.7341045267725,-10.4006828199142));
#41651=CARTESIAN_POINT('Ctrl Pts',(-18.1723394871415,16.711817262327,-10.4050692819268));
#41652=CARTESIAN_POINT('Ctrl Pts',(-18.2587188895798,16.6939693367971,-10.4094557439393));
#41653=CARTESIAN_POINT('Ctrl Pts',(-18.3456526669335,16.6806272312364,-10.4138422059519));
#41654=CARTESIAN_POINT('Ctrl Pts',(-18.4325864442873,16.6672851256758,-10.4182286679644));
#41655=CARTESIAN_POINT('Ctrl Pts',(-18.5200740116326,16.6584488227101,-10.422615129977));
#41656=CARTESIAN_POINT('Ctrl Pts',(-18.6076132463768,16.6541217493771,-10.4270015919895));
#41657=CARTESIAN_POINT('Ctrl Pts',(-18.6911246711663,16.6499937711024,-10.4311862263825));
#41658=CARTESIAN_POINT('Ctrl Pts',(-18.7749939587051,16.6499538232249,-10.4353708607756));
#41659=CARTESIAN_POINT('Ctrl Pts',(-18.8587871646375,16.6540431830902,-10.4395554951686));
#41660=CARTESIAN_POINT('Ctrl Pts',(-18.9424611013126,16.6581267222578,-10.4437341732526));
#41661=CARTESIAN_POINT('Ctrl Pts',(-19.0260587159288,16.6663278722549,-10.4479128513365));
#41662=CARTESIAN_POINT('Ctrl Pts',(-19.1091432618588,16.6786359793502,-10.4520915294204));
#41663=CARTESIAN_POINT('Ctrl Pts',(-19.1937170385631,16.6911647004194,-10.4563451073059));
#41664=CARTESIAN_POINT('Ctrl Pts',(-19.2777586905999,16.7079490849926,-10.4605986851913));
#41665=CARTESIAN_POINT('Ctrl Pts',(-19.360809982363,16.7289223932338,-10.4648522630768));
#41666=CARTESIAN_POINT('Ctrl Pts',(-19.4422511627741,16.7494890929688,-10.4690233770547));
#41667=CARTESIAN_POINT('Ctrl Pts',(-19.5227395737969,16.7740836270436,-10.4731944910327));
#41668=CARTESIAN_POINT('Ctrl Pts',(-19.6018523684377,16.8025913414462,-10.4773656050106));
#41669=CARTESIAN_POINT('Ctrl Pts',(-19.6809386160161,16.8310894898098,-10.481535319331));
#41670=CARTESIAN_POINT('Ctrl Pts',(-19.7586497315284,16.8634980548293,-10.4857050336514));
#41671=CARTESIAN_POINT('Ctrl Pts',(-19.8345791893309,16.8996528932219,-10.4898747479717));
#41672=CARTESIAN_POINT('Ctrl Pts',(-19.9105059452373,16.93580644507,-10.4940443139158));
#41673=CARTESIAN_POINT('Ctrl Pts',(-19.984650754504,16.9757058066958,-10.4982138798598));
#41674=CARTESIAN_POINT('Ctrl Pts',(-20.0566294498833,17.0191397539302,-10.5023834458038));
#41675=CARTESIAN_POINT('Ctrl Pts',(-20.131138827397,17.0641007851678,-10.5066996085427));
#41676=CARTESIAN_POINT('Ctrl Pts',(-20.2033264842377,17.1128493061259,-10.5110157712817));
#41677=CARTESIAN_POINT('Ctrl Pts',(-20.2727983186242,17.1651017291666,-10.5153319340206));
#41678=CARTESIAN_POINT('Ctrl Pts',(-20.3400071153126,17.2156520350226,-10.5195074982123));
#41679=CARTESIAN_POINT('Ctrl Pts',(-20.4046739763887,17.2694811317351,-10.5236830624039));
#41680=CARTESIAN_POINT('Ctrl Pts',(-20.4664767307265,17.326291964921,-10.5278586265956));
#41681=CARTESIAN_POINT('Ctrl Pts',(-20.5314009952638,17.3859721782363,-10.5322450886082));
#41682=CARTESIAN_POINT('Ctrl Pts',(-20.593163808364,17.4489428422735,-10.5366315506207));
#41683=CARTESIAN_POINT('Ctrl Pts',(-20.6514380125587,17.5148185627725,-10.5410180126333));
#41684=CARTESIAN_POINT('Ctrl Pts',(-20.7097122167533,17.5806942832716,-10.5454044746458));
#41685=CARTESIAN_POINT('Ctrl Pts',(-20.7644975100434,17.6494745589998,-10.5497909366583));
#41686=CARTESIAN_POINT('Ctrl Pts',(-20.8155192213964,17.7207390393097,-10.5541773986709));
#41687=CARTESIAN_POINT('Ctrl Pts',(-20.8646271615162,17.789330463214,-10.5583993290636));
#41688=CARTESIAN_POINT('Ctrl Pts',(-20.91043082465,17.8604769154309,-10.5626212594563));
#41689=CARTESIAN_POINT('Ctrl Pts',(-20.9526566798058,17.9338302629825,-10.5668431898491));
#41690=CARTESIAN_POINT('Ctrl Pts',(-20.9948201353165,18.0070752119515,-10.5710588812454));
#41691=CARTESIAN_POINT('Ctrl Pts',(-21.0334160638336,18.0825201920568,-10.5752745726417));
#41692=CARTESIAN_POINT('Ctrl Pts',(-21.0682129788551,18.1597865253222,-10.5794902640381));
#41693=CARTESIAN_POINT('Ctrl Pts',(-21.1029682787106,18.2369604523702,-10.583700913703));
#41694=CARTESIAN_POINT('Ctrl Pts',(-21.1339334100817,18.3159509969196,-10.587911563368));
#41695=CARTESIAN_POINT('Ctrl Pts',(-21.1609223976387,18.3963542635971,-10.592122213033));
#41696=CARTESIAN_POINT('Ctrl Pts',(-21.1878844462894,18.4766772762055,-10.5963286598616));
#41697=CARTESIAN_POINT('Ctrl Pts',(-21.2108781024617,18.5584097818782,-10.6005351066903));
#41698=CARTESIAN_POINT('Ctrl Pts',(-21.2297657078559,18.6411284956323,-10.6047415535189));
#41699=CARTESIAN_POINT('Ctrl Pts',(-21.24864245849,18.7237996707081,-10.6089455828907));
#41700=CARTESIAN_POINT('Ctrl Pts',(-21.2634177498248,18.8074554899473,-10.6131496122625));
#41701=CARTESIAN_POINT('Ctrl Pts',(-21.2740042132099,18.8916591211951,-10.6173536416343));
#41702=CARTESIAN_POINT('Ctrl Pts',(-21.2845883389273,18.975844158876,-10.6215567426862));
#41703=CARTESIAN_POINT('Ctrl Pts',(-21.2909854180498,19.0605763228041,-10.6257598437382));
#41704=CARTESIAN_POINT('Ctrl Pts',(-21.2931596531403,19.1454113596826,-10.6299629447901));
#41705=CARTESIAN_POINT('Ctrl Pts',(-21.2937333596144,19.1677964320698,-10.6310719997839));
#41706=CARTESIAN_POINT('Ctrl Pts',(-21.2940133304248,19.1901886456573,-10.6321810547777));
#41707=CARTESIAN_POINT('Ctrl Pts',(-21.2939995125392,19.2125798097912,-10.6332901097715));
#41708=CARTESIAN_POINT('Ctrl Pts',(-21.2907953051338,19.2125971079063,-10.6332910656997));
#41709=CARTESIAN_POINT('Ctrl Pts',(-21.292607272731,19.5356421908361,-10.6493117789173));
#41710=CARTESIAN_POINT('Ctrl Pts',(-21.0857646549701,20.7112479426697,-10.7077244276952));
#41711=CARTESIAN_POINT('Ctrl Pts',(-19.4306371445278,22.0881475490561,-10.8021586269852));
#41712=CARTESIAN_POINT('Ctrl Pts',(-17.7502563260471,21.6776341328961,-10.8805721130576));
#41713=CARTESIAN_POINT('Ctrl Pts',(-17.173194974388,21.2428171613069,-10.9165936635695));
#41714=CARTESIAN_POINT('',(-21.2940196853139,19.2096989556262,-10.5667098967305));
#41715=CARTESIAN_POINT('Ctrl Pts',(-21.2974135715529,19.2097193143547,-10.5667109992077));
#41716=CARTESIAN_POINT('Ctrl Pts',(-21.292595768045,19.9846331911651,-10.6053965865519));
#41717=CARTESIAN_POINT('Ctrl Pts',(-20.5048168766745,21.6171665132323,-10.6864741094567));
#41718=CARTESIAN_POINT('Ctrl Pts',(-18.3777720364044,21.9601260692161,-10.7809759372829));
#41719=CARTESIAN_POINT('Ctrl Pts',(-17.3887251838872,21.4060795618296,-10.8367921777649));
#41720=CARTESIAN_POINT('Ctrl Pts',(-17.1757181329864,21.2395346319229,-10.8502164826864));
#41721=CARTESIAN_POINT('Ctrl Pts',(-17.1744642439897,21.2411350264762,-10.0501312698105));
#41722=CARTESIAN_POINT('Ctrl Pts',(-17.1081216278261,21.1901710853072,-10.0543142329175));
#41723=CARTESIAN_POINT('Ctrl Pts',(-17.0441628085899,21.1358618379643,-10.0584971960246));
#41724=CARTESIAN_POINT('Ctrl Pts',(-16.9829440292627,21.0784589653712,-10.0626801591317));
#41725=CARTESIAN_POINT('Ctrl Pts',(-16.9218071503208,21.0211328881247,-10.0668575261407));
#41726=CARTESIAN_POINT('Ctrl Pts',(-16.8634033625468,20.9607217193491,-10.0710348931497));
#41727=CARTESIAN_POINT('Ctrl Pts',(-16.8080571271221,20.8975183219908,-10.0752122601588));
#41728=CARTESIAN_POINT('Ctrl Pts',(-16.7527685070128,20.834380719237,-10.0793852785375));
#41729=CARTESIAN_POINT('Ctrl Pts',(-16.7005314148742,20.7684570095275,-10.0835582969162));
#41730=CARTESIAN_POINT('Ctrl Pts',(-16.6516336173591,20.700076978684,-10.0877313152949));
#41731=CARTESIAN_POINT('Ctrl Pts',(-16.6027633898385,20.6317355024826,-10.091901980805));
#41732=CARTESIAN_POINT('Ctrl Pts',(-16.5572289858127,20.5609408282047,-10.0960726463151));
#41733=CARTESIAN_POINT('Ctrl Pts',(-16.5152772819117,20.4880550106548,-10.1002433118252));
#41734=CARTESIAN_POINT('Ctrl Pts',(-16.4733366469514,20.4151884239997,-10.1044128769068));
#41735=CARTESIAN_POINT('Ctrl Pts',(-16.4349770638098,20.3402321885223,-10.1085824419884));
#41736=CARTESIAN_POINT('Ctrl Pts',(-16.4004007975782,20.2635753001359,-10.11275200707));
#41737=CARTESIAN_POINT('Ctrl Pts',(-16.365823282296,20.1869156425573,-10.1169217227751));
#41738=CARTESIAN_POINT('Ctrl Pts',(-16.3350295432698,20.1085556299752,-10.1210914384802));
#41739=CARTESIAN_POINT('Ctrl Pts',(-16.3081742243601,20.0289054384468,-10.1252611541852));
#41740=CARTESIAN_POINT('Ctrl Pts',(-16.2812914480234,19.9491738109349,-10.1294351330929));
#41741=CARTESIAN_POINT('Ctrl Pts',(-16.2583552817622,19.8681498067063,-10.1336091120005));
#41742=CARTESIAN_POINT('Ctrl Pts',(-16.2394706988067,19.786259563578,-10.1377830909082));
#41743=CARTESIAN_POINT('Ctrl Pts',(-16.2205765762285,19.7043279532655,-10.141959178318));
#41744=CARTESIAN_POINT('Ctrl Pts',(-16.2057381946938,19.6215296857435,-10.1461352657278));
#41745=CARTESIAN_POINT('Ctrl Pts',(-16.1950090508136,19.5382994957977,-10.1503113531375));
#41746=CARTESIAN_POINT('Ctrl Pts',(-16.1842607922711,19.4549210258973,-10.1544948805166));
#41747=CARTESIAN_POINT('Ctrl Pts',(-16.1776364344997,19.3711095556487,-10.1586784078956));
#41748=CARTESIAN_POINT('Ctrl Pts',(-16.1751373971613,19.2873032095876,-10.1628619352746));
#41749=CARTESIAN_POINT('Ctrl Pts',(-16.1729067664636,19.2124980014741,-10.1665961350213));
#41750=CARTESIAN_POINT('Ctrl Pts',(-16.1739621448211,19.1376971079801,-10.170330334768));
#41751=CARTESIAN_POINT('Ctrl Pts',(-16.1782696504243,19.0632083214198,-10.1740645345148));
#41752=CARTESIAN_POINT('Ctrl Pts',(-16.1830967452018,18.9797343887762,-10.1782491689078));
#41753=CARTESIAN_POINT('Ctrl Pts',(-16.1920266966377,18.8963418534062,-10.1824338033009));
#41754=CARTESIAN_POINT('Ctrl Pts',(-16.205054135763,18.8134665853562,-10.1866184376939));
#41755=CARTESIAN_POINT('Ctrl Pts',(-16.2180630319411,18.7307092799923,-10.1907971157779));
#41756=CARTESIAN_POINT('Ctrl Pts',(-16.2351577602661,18.648468230058,-10.1949757938618));
#41757=CARTESIAN_POINT('Ctrl Pts',(-16.2562810188397,18.567176537863,-10.1991544719458));
#41758=CARTESIAN_POINT('Ctrl Pts',(-16.2777828966423,18.4844277505086,-10.2034080498312));
#41759=CARTESIAN_POINT('Ctrl Pts',(-16.3034591202047,18.4026631714652,-10.2076616277166));
#41760=CARTESIAN_POINT('Ctrl Pts',(-16.3331943249929,18.322331270465,-10.2119152056021));
#41761=CARTESIAN_POINT('Ctrl Pts',(-16.3623530548127,18.2435567601205,-10.21608631958));
#41762=CARTESIAN_POINT('Ctrl Pts',(-16.3954146207213,18.1661603243175,-10.220257433558));
#41763=CARTESIAN_POINT('Ctrl Pts',(-16.4322198035646,18.0905501228088,-10.2244285475359));
#41764=CARTESIAN_POINT('Ctrl Pts',(-16.4690126360733,18.0149652930334,-10.2285982618563));
#41765=CARTESIAN_POINT('Ctrl Pts',(-16.5095463894924,17.9411659204443,-10.2327679761767));
#41766=CARTESIAN_POINT('Ctrl Pts',(-16.5536143847776,17.8695386442647,-10.236937690497));
#41767=CARTESIAN_POINT('Ctrl Pts',(-16.5976808119345,17.7979139168909,-10.2411072564411));
#41768=CARTESIAN_POINT('Ctrl Pts',(-16.6452809891205,17.7284615236186,-10.2452768223851));
#41769=CARTESIAN_POINT('Ctrl Pts',(-16.6961638176235,17.6615408382932,-10.2494463883292));
#41770=CARTESIAN_POINT('Ctrl Pts',(-16.7488356236059,17.5922673042274,-10.2537625510681));
#41771=CARTESIAN_POINT('Ctrl Pts',(-16.8050248926421,17.5257072400677,-10.258078713807));
#41772=CARTESIAN_POINT('Ctrl Pts',(-16.8644075151044,17.462222158071,-10.2623948765459));
#41773=CARTESIAN_POINT('Ctrl Pts',(-16.9218557548859,17.4008050959429,-10.2665704407376));
#41774=CARTESIAN_POINT('Ctrl Pts',(-16.9822921248588,17.3422660512049,-10.2707460049293));
#41775=CARTESIAN_POINT('Ctrl Pts',(-17.0453868187423,17.2868935777658,-10.274921569121));
#41776=CARTESIAN_POINT('Ctrl Pts',(-17.1116682756205,17.2287243723289,-10.2793080311335));
#41777=CARTESIAN_POINT('Ctrl Pts',(-17.1808831995726,17.1740503939332,-10.283694493146));
#41778=CARTESIAN_POINT('Ctrl Pts',(-17.2526134178259,17.1231557064392,-10.2880809551586));
#41779=CARTESIAN_POINT('Ctrl Pts',(-17.3243436360791,17.0722610189452,-10.2924674171711));
#41780=CARTESIAN_POINT('Ctrl Pts',(-17.3985886179775,17.0251458690142,-10.2968538791837));
#41781=CARTESIAN_POINT('Ctrl Pts',(-17.4749010481802,16.9820383965787,-10.3012403411962));
#41782=CARTESIAN_POINT('Ctrl Pts',(-17.5477022303472,16.9409143628506,-10.3054249755892));
#41783=CARTESIAN_POINT('Ctrl Pts',(-17.6226557687809,16.9032842410815,-10.3096096099823));
#41784=CARTESIAN_POINT('Ctrl Pts',(-17.6993922596291,16.8693794450073,-10.3137942443753));
#41785=CARTESIAN_POINT('Ctrl Pts',(-17.7760195255806,16.8355229082136,-10.3179729224593));
#41786=CARTESIAN_POINT('Ctrl Pts',(-17.8544242858621,16.8053813489309,-10.3221516005432));
#41787=CARTESIAN_POINT('Ctrl Pts',(-17.9342113535406,16.779141015397,-10.3263302786272));
#41788=CARTESIAN_POINT('Ctrl Pts',(-18.0154285470652,16.752430342743,-10.3305838565126));
#41789=CARTESIAN_POINT('Ctrl Pts',(-18.0980776713418,16.7297623675601,-10.334837434398));
#41790=CARTESIAN_POINT('Ctrl Pts',(-18.1817191896631,16.7112828346924,-10.3390910122835));
#41791=CARTESIAN_POINT('Ctrl Pts',(-18.2637391539388,16.6931615636291,-10.3432621262614));
#41792=CARTESIAN_POINT('Ctrl Pts',(-18.3467129067616,16.6790678856914,-10.3474332402394));
#41793=CARTESIAN_POINT('Ctrl Pts',(-18.4302110680642,16.6690888519004,-10.3516043542173));
#41794=CARTESIAN_POINT('Ctrl Pts',(-18.5136812107523,16.6591131666705,-10.3557740685377));
#41795=CARTESIAN_POINT('Ctrl Pts',(-18.5976749560381,16.6532494380237,-10.3599437828581));
#41796=CARTESIAN_POINT('Ctrl Pts',(-18.6817553300752,16.6515331620698,-10.3641134971784));
#41797=CARTESIAN_POINT('Ctrl Pts',(-18.7658327121718,16.6498169471884,-10.3682830631225));
#41798=CARTESIAN_POINT('Ctrl Pts',(-18.8499962569362,16.652247900101,-10.3724526290665));
#41799=CARTESIAN_POINT('Ctrl Pts',(-18.9338078728663,16.6588094087744,-10.3766221950106));
#41800=CARTESIAN_POINT('Ctrl Pts',(-19.0205662018197,16.6656016119982,-10.3809383577495));
#41801=CARTESIAN_POINT('Ctrl Pts',(-19.1069468680349,16.6768201947949,-10.3852545204884));
#41802=CARTESIAN_POINT('Ctrl Pts',(-19.1924704625205,16.6923883119869,-10.3895706832273));
#41803=CARTESIAN_POINT('Ctrl Pts',(-19.2752081349112,16.7074492993989,-10.393746247419));
#41804=CARTESIAN_POINT('Ctrl Pts',(-19.357143268331,16.7265806476473,-10.3979218116107));
#41805=CARTESIAN_POINT('Ctrl Pts',(-19.437854716723,16.749661230601,-10.4020973758024));
#41806=CARTESIAN_POINT('Ctrl Pts',(-19.5226427085001,16.7739075589308,-10.4064838378149));
#41807=CARTESIAN_POINT('Ctrl Pts',(-19.6060795975567,16.8025123689437,-10.4108702998274));
#41808=CARTESIAN_POINT('Ctrl Pts',(-19.6877001821495,16.8352778018952,-10.41525676184));
#41809=CARTESIAN_POINT('Ctrl Pts',(-19.7693207667423,16.8680432348467,-10.4196432238525));
#41810=CARTESIAN_POINT('Ctrl Pts',(-19.8491245522344,16.9049689780518,-10.4240296858651));
#41811=CARTESIAN_POINT('Ctrl Pts',(-19.9266775857362,16.945802397917,-10.4284161478776));
#41812=CARTESIAN_POINT('Ctrl Pts',(-20.0006622892055,16.9847570116046,-10.4326007822707));
#41813=CARTESIAN_POINT('Ctrl Pts',(-20.0728741952653,17.0274126045708,-10.4367854166637));
#41814=CARTESIAN_POINT('Ctrl Pts',(-20.1429187702869,17.0735838265015,-10.4409700510568));
#41815=CARTESIAN_POINT('Ctrl Pts',(-20.2128636455258,17.1196893294125,-10.4451487291407));
#41816=CARTESIAN_POINT('Ctrl Pts',(-20.2806469365539,17.1693002706272,-10.4493274072247));
#41817=CARTESIAN_POINT('Ctrl Pts',(-20.3458981308861,17.2221851731129,-10.4535060853086));
#41818=CARTESIAN_POINT('Ctrl Pts',(-20.4123189059815,17.276017999468,-10.457759663194));
#41819=CARTESIAN_POINT('Ctrl Pts',(-20.4761154892317,17.3332430884428,-10.4620132410795));
#41820=CARTESIAN_POINT('Ctrl Pts',(-20.5369274194045,17.3935697481445,-10.4662668189649));
#41821=CARTESIAN_POINT('Ctrl Pts',(-20.5965603916461,17.4527268578301,-10.4704379329429));
#41822=CARTESIAN_POINT('Ctrl Pts',(-20.6533230631002,17.5148660125131,-10.4746090469208));
#41823=CARTESIAN_POINT('Ctrl Pts',(-20.7069098223473,17.5796732905743,-10.4787801608988));
#41824=CARTESIAN_POINT('Ctrl Pts',(-20.7604786000398,17.6444588219275,-10.4829498752191));
#41825=CARTESIAN_POINT('Ctrl Pts',(-20.8108732891324,17.7119103443124,-10.4871195895395));
#41826=CARTESIAN_POINT('Ctrl Pts',(-20.857827517359,17.7816796452479,-10.4912893038599));
#41827=CARTESIAN_POINT('Ctrl Pts',(-20.9047800747525,17.8514464634921,-10.4954588698039));
#41828=CARTESIAN_POINT('Ctrl Pts',(-20.9482921585527,17.9235305141741,-10.499628435748));
#41829=CARTESIAN_POINT('Ctrl Pts',(-20.9881406062296,17.9975544398916,-10.503798001692));
#41830=CARTESIAN_POINT('Ctrl Pts',(-21.0293900761685,18.074180955519,-10.5081141644309));
#41831=CARTESIAN_POINT('Ctrl Pts',(-21.0667132396991,18.1528858318598,-10.5124303271698));
#41832=CARTESIAN_POINT('Ctrl Pts',(-21.0999152164604,18.2332243669833,-10.5167464899088));
#41833=CARTESIAN_POINT('Ctrl Pts',(-21.1320356423208,18.3109458827751,-10.5209220541004));
#41834=CARTESIAN_POINT('Ctrl Pts',(-21.1602991397429,18.3901957994174,-10.5250976182921));
#41835=CARTESIAN_POINT('Ctrl Pts',(-21.1845795982611,18.4705544364463,-10.5292731824838));
#41836=CARTESIAN_POINT('Ctrl Pts',(-21.2100864050179,18.5549717971972,-10.5336596444963));
#41837=CARTESIAN_POINT('Ctrl Pts',(-21.2311970921469,18.6406122578467,-10.5380461065089));
#41838=CARTESIAN_POINT('Ctrl Pts',(-21.2478262226602,18.7269775601629,-10.5424325685214));
#41839=CARTESIAN_POINT('Ctrl Pts',(-21.2644553531735,18.813342862479,-10.5468190305339));
#41840=CARTESIAN_POINT('Ctrl Pts',(-21.2766029222518,18.9004324212998,-10.5512054925465));
#41841=CARTESIAN_POINT('Ctrl Pts',(-21.2842464642989,18.9877446051473,-10.555591954559));
#41842=CARTESIAN_POINT('Ctrl Pts',(-21.2907042434478,19.0615118189368,-10.5592979331155));
#41843=CARTESIAN_POINT('Ctrl Pts',(-21.293961988618,19.1355632322755,-10.563003911672));
#41844=CARTESIAN_POINT('Ctrl Pts',(-21.2939996693303,19.2096988355573,-10.5667098902285));
#41845=CARTESIAN_POINT('Origin',(-18.734,19.211,1.76670989022852));
#41846=CARTESIAN_POINT('',(-17.1744642439897,21.2411350264762,-9.25004023969327));
#41847=CARTESIAN_POINT('',(-17.1750494706851,21.2403917593384,-9.31680760799386));
#41848=CARTESIAN_POINT('',(-17.1744642439897,21.2411350264762,1.76670989022852));
#41849=CARTESIAN_POINT('',(-21.2939992159918,19.2089964727374,-9.8332901097715));
#41850=CARTESIAN_POINT('Ctrl Pts',(-17.1750494706848,21.2403917593382,-9.31680760799388));
#41851=CARTESIAN_POINT('Ctrl Pts',(-16.6852502113565,20.8565255580946,-9.34773678484192));
#41852=CARTESIAN_POINT('Ctrl Pts',(-15.8397229750276,19.5224826623952,-9.42105789725044));
#41853=CARTESIAN_POINT('Ctrl Pts',(-16.6528318707067,17.0128118877737,-9.53677094521943));
#41854=CARTESIAN_POINT('Ctrl Pts',(-19.4558314956606,16.2712294220481,-9.66394675190088));
#41855=CARTESIAN_POINT('Ctrl Pts',(-21.1196060595483,17.7909993809188,-9.76278617061903));
#41856=CARTESIAN_POINT('Ctrl Pts',(-21.2937097337482,18.9257985538188,-9.81923365377672));
#41857=CARTESIAN_POINT('Ctrl Pts',(-21.2916489871171,19.2089800104295,-9.83328920137392));
#41858=CARTESIAN_POINT('Ctrl Pts',(-21.2939992159918,19.2089964727374,-9.8332901097715));
#41859=CARTESIAN_POINT('Ctrl Pts',(-21.2940649620946,19.2930033015151,-9.83745593779552));
#41860=CARTESIAN_POINT('Ctrl Pts',(-21.2899913508454,19.3770604200798,-9.84162176581953));
#41861=CARTESIAN_POINT('Ctrl Pts',(-21.281790209728,19.4607299485725,-9.84578759384355));
#41862=CARTESIAN_POINT('Ctrl Pts',(-21.2735905258927,19.544384609609,-9.84995268163075));
#41863=CARTESIAN_POINT('Ctrl Pts',(-21.2612648140692,19.6276513592372,-9.85411776941795));
#41864=CARTESIAN_POINT('Ctrl Pts',(-21.2448768408732,19.7100966739687,-9.85828285720515));
#41865=CARTESIAN_POINT('Ctrl Pts',(-21.2284868533627,19.7925521223993,-9.86244845694073));
#41866=CARTESIAN_POINT('Ctrl Pts',(-21.2080337038204,19.8741854840197,-9.86661405667632));
#41867=CARTESIAN_POINT('Ctrl Pts',(-21.183632148948,19.9545740278144,-9.8707796564119));
#41868=CARTESIAN_POINT('Ctrl Pts',(-21.159203008195,20.0350534506039,-9.87494996534483));
#41869=CARTESIAN_POINT('Ctrl Pts',(-21.1308166833999,20.114284804087,-9.87912027427776));
#41870=CARTESIAN_POINT('Ctrl Pts',(-21.0986375209739,20.1918615572049,-9.88329058321069));
#41871=CARTESIAN_POINT('Ctrl Pts',(-21.066439637101,20.2694834435379,-9.88746331837884));
#41872=CARTESIAN_POINT('Ctrl Pts',(-21.0304447198545,20.3454483968716,-9.89163605354698));
#41873=CARTESIAN_POINT('Ctrl Pts',(-20.9908638255709,20.4193731513193,-9.89580878871513));
#41874=CARTESIAN_POINT('Ctrl Pts',(-20.9512104382913,20.4934333000532,-9.89998916630974));
#41875=CARTESIAN_POINT('Ctrl Pts',(-20.907958193034,20.5654453913561,-9.90416954390436));
#41876=CARTESIAN_POINT('Ctrl Pts',(-20.8613622504221,20.6350540212643,-9.90834992149897));
#41877=CARTESIAN_POINT('Ctrl Pts',(-20.8243993123263,20.6902721225411,-9.91166606942056));
#41878=CARTESIAN_POINT('Ctrl Pts',(-20.7853331875374,20.7439783287845,-9.91498221734216));
#41879=CARTESIAN_POINT('Ctrl Pts',(-20.7443085775785,20.7960108589263,-9.91829836526375));
#41880=CARTESIAN_POINT('Ctrl Pts',(-20.6925397790042,20.8616705099241,-9.9224829996568));
#41881=CARTESIAN_POINT('Ctrl Pts',(-20.6374544461771,20.9249134154189,-9.92666763404984));
#41882=CARTESIAN_POINT('Ctrl Pts',(-20.5793066365797,20.9853853631595,-9.93085226844289));
#41883=CARTESIAN_POINT('Ctrl Pts',(-20.5212415931921,21.0457712365674,-9.93503094652683));
#41884=CARTESIAN_POINT('Ctrl Pts',(-20.4601230476226,21.1033936577093,-9.93920962461076));
#41885=CARTESIAN_POINT('Ctrl Pts',(-20.3962460420505,21.1579304290825,-9.9433883026947));
#41886=CARTESIAN_POINT('Ctrl Pts',(-20.3312240870609,21.2134447328878,-9.94764188058014));
#41887=CARTESIAN_POINT('Ctrl Pts',(-20.2633441071063,21.2657612997089,-9.95189545846558));
#41888=CARTESIAN_POINT('Ctrl Pts',(-20.1929575410587,21.3145785921586,-9.95614903635102));
#41889=CARTESIAN_POINT('Ctrl Pts',(-20.1239355559419,21.3624494661351,-9.96032015032897));
#41890=CARTESIAN_POINT('Ctrl Pts',(-20.0525037029722,21.4069552612257,-9.96449126430692));
#41891=CARTESIAN_POINT('Ctrl Pts',(-19.979026280494,21.4478526015094,-9.96866237828488));
#41892=CARTESIAN_POINT('Ctrl Pts',(-19.9055735140746,21.4887362182955,-9.97283209260525));
#41893=CARTESIAN_POINT('Ctrl Pts',(-19.8300769429976,21.5260135615003,-9.97700180692563));
#41894=CARTESIAN_POINT('Ctrl Pts',(-19.7529274425308,21.5594860797666,-9.981171521246));
#41895=CARTESIAN_POINT('Ctrl Pts',(-19.6757806873742,21.5929574069372,-9.98534108719005));
#41896=CARTESIAN_POINT('Ctrl Pts',(-19.5969815421365,21.6226239960434,-9.98951065313409));
#41897=CARTESIAN_POINT('Ctrl Pts',(-19.5169416763859,21.6483350880373,-9.99368021907814));
#41898=CARTESIAN_POINT('Ctrl Pts',(-19.4340877076953,21.6749501503077,-9.99799638181706));
#41899=CARTESIAN_POINT('Ctrl Pts',(-19.3499046498555,21.6973262283484,-10.002312544556));
#41900=CARTESIAN_POINT('Ctrl Pts',(-19.264865245119,21.7153526292287,-10.0066287072949));
#41901=CARTESIAN_POINT('Ctrl Pts',(-19.1825959900473,21.7327918219964,-10.0108042714866));
#41902=CARTESIAN_POINT('Ctrl Pts',(-19.0995257948678,21.7461603390116,-10.0149798356783));
#41903=CARTESIAN_POINT('Ctrl Pts',(-19.0160902825554,21.7554105550182,-10.0191553998699));
#41904=CARTESIAN_POINT('Ctrl Pts',(-18.9284406408651,21.7651279774449,-10.0235418618825));
#41905=CARTESIAN_POINT('Ctrl Pts',(-18.840388390719,21.7703001003684,-10.027928323895));
#41906=CARTESIAN_POINT('Ctrl Pts',(-18.7524390182804,21.7709335933975,-10.0323147859076));
#41907=CARTESIAN_POINT('Ctrl Pts',(-18.6644896458417,21.7715670864265,-10.0367012479201));
#41908=CARTESIAN_POINT('Ctrl Pts',(-18.576643727377,21.767662051318,-10.0410877099326));
#41909=CARTESIAN_POINT('Ctrl Pts',(-18.4893986055751,21.759287691342,-10.0454741719452));
#41910=CARTESIAN_POINT('Ctrl Pts',(-18.4061740830914,21.7512992549033,-10.0496584884874));
#41911=CARTESIAN_POINT('Ctrl Pts',(-18.3231864480374,21.7392146225049,-10.0538428050297));
#41912=CARTESIAN_POINT('Ctrl Pts',(-18.2408709541661,21.7230556809424,-10.058027121572));
#41913=CARTESIAN_POINT('Ctrl Pts',(-18.1586671961938,21.7069186736935,-10.0622057582799));
#41914=CARTESIAN_POINT('Ctrl Pts',(-18.0771342151523,21.6867184269545,-10.0663843949878));
#41915=CARTESIAN_POINT('Ctrl Pts',(-17.9967026166128,21.6625286187296,-10.0705630316957));
#41916=CARTESIAN_POINT('Ctrl Pts',(-17.9163646373026,21.6383669664937,-10.0747368046342));
#41917=CARTESIAN_POINT('Ctrl Pts',(-17.8371259304894,21.6102251148538,-10.0789105775727));
#41918=CARTESIAN_POINT('Ctrl Pts',(-17.75940588948,21.578227559771,-10.0830843505111));
#41919=CARTESIAN_POINT('Ctrl Pts',(-17.6817391959917,21.5462519680098,-10.0872552585458));
#41920=CARTESIAN_POINT('Ctrl Pts',(-17.6055895218583,21.5104261042808,-10.0914261665805));
#41921=CARTESIAN_POINT('Ctrl Pts',(-17.531359015293,21.4709235964746,-10.0955970746152));
#41922=CARTESIAN_POINT('Ctrl Pts',(-17.4571459112369,21.4314303495882,-10.0997670048274));
#41923=CARTESIAN_POINT('Ctrl Pts',(-17.3848514901506,21.3882623802804,-10.1039369350395));
#41924=CARTESIAN_POINT('Ctrl Pts',(-17.3148548334226,21.341640043785,-10.1081068652516));
#41925=CARTESIAN_POINT('Ctrl Pts',(-17.266943957738,21.3097282772467,-10.1109610731144));
#41926=CARTESIAN_POINT('Ctrl Pts',(-17.2201091169427,21.276199103752,-10.1138152809773));
#41927=CARTESIAN_POINT('Ctrl Pts',(-17.1744642439897,21.2411350264762,-10.1166694888401));
#41928=CARTESIAN_POINT('',(-21.2939989766127,19.2132890482675,-9.7667098901893));
#41929=CARTESIAN_POINT('Ctrl Pts',(-21.293998976612,19.2132890490549,-9.76670989022852));
#41930=CARTESIAN_POINT('Ctrl Pts',(-21.2938920610985,19.3328599270272,-9.77266511192853));
#41931=CARTESIAN_POINT('Ctrl Pts',(-21.2854044483393,19.4520702292311,-9.77862033362855));
#41932=CARTESIAN_POINT('Ctrl Pts',(-21.2687069780215,19.5699714968758,-9.78457555532857));
#41933=CARTESIAN_POINT('Ctrl Pts',(-21.2612660069347,19.6225123852221,-9.78722940837586));
#41934=CARTESIAN_POINT('Ctrl Pts',(-21.2521952261605,19.6747937484515,-9.78988326142315));
#41935=CARTESIAN_POINT('Ctrl Pts',(-21.2415125421986,19.7267333135613,-9.79253711447044));
#41936=CARTESIAN_POINT('Ctrl Pts',(-21.2246679295087,19.8086323813113,-9.79672174886349));
#41937=CARTESIAN_POINT('Ctrl Pts',(-21.2037753333228,19.8898577370366,-9.80090638325654));
#41938=CARTESIAN_POINT('Ctrl Pts',(-21.1789030820534,19.9699788662181,-9.80509101764959));
#41939=CARTESIAN_POINT('Ctrl Pts',(-21.154066233355,20.0499859528893,-9.80926969573354));
#41940=CARTESIAN_POINT('Ctrl Pts',(-21.125261116367,20.1288914993745,-9.81344837381749));
#41941=CARTESIAN_POINT('Ctrl Pts',(-21.0926070466711,20.2062752380087,-9.81762705190143));
#41942=CARTESIAN_POINT('Ctrl Pts',(-21.0593676762441,20.2850460245431,-9.82188062978687));
#41943=CARTESIAN_POINT('Ctrl Pts',(-21.022140108072,20.362239437543,-9.8261342076723));
#41944=CARTESIAN_POINT('Ctrl Pts',(-20.9811033321017,20.4374283977703,-9.83038778555774));
#41945=CARTESIAN_POINT('Ctrl Pts',(-20.9408621341102,20.5111596732845,-9.83455889953569));
#41946=CARTESIAN_POINT('Ctrl Pts',(-20.8969583386824,20.5829631005171,-9.83873001351364));
#41947=CARTESIAN_POINT('Ctrl Pts',(-20.8496085018329,20.6524578269836,-9.84290112749159));
#41948=CARTESIAN_POINT('Ctrl Pts',(-20.8022745536785,20.7219292338234,-9.84707084181197));
#41949=CARTESIAN_POINT('Ctrl Pts',(-20.7514971194517,20.7890930986179,-9.85124055613234));
#41950=CARTESIAN_POINT('Ctrl Pts',(-20.6975366051101,20.853596724821,-9.85541027045272));
#41951=CARTESIAN_POINT('Ctrl Pts',(-20.643578010915,20.9180980557084,-9.85957983639676));
#41952=CARTESIAN_POINT('Ctrl Pts',(-20.5864368576391,20.9799389839169,-9.86374940234081));
#41953=CARTESIAN_POINT('Ctrl Pts',(-20.5264135623405,21.0388002137919,-9.86791896828486));
#41954=CARTESIAN_POINT('Ctrl Pts',(-20.4642799220261,21.099730931896,-9.87223513102378));
#41955=CARTESIAN_POINT('Ctrl Pts',(-20.3990580731255,21.1574681514492,-9.87655129376269));
#41956=CARTESIAN_POINT('Ctrl Pts',(-20.3311209857105,21.2117010163947,-9.88086745650161));
#41957=CARTESIAN_POINT('Ctrl Pts',(-20.2653969417723,21.264167251469,-9.88504302069329));
#41958=CARTESIAN_POINT('Ctrl Pts',(-20.1971322502975,21.3133536974901,-9.88921858488498));
#41959=CARTESIAN_POINT('Ctrl Pts',(-20.1266949702183,21.3590225138319,-9.89339414907666));
#41960=CARTESIAN_POINT('Ctrl Pts',(-20.0527000705711,21.4069979535197,-9.89778061108919));
#41961=CARTESIAN_POINT('Ctrl Pts',(-19.9763078452047,21.4510907819034,-9.90216707310173));
#41962=CARTESIAN_POINT('Ctrl Pts',(-19.8979731420051,21.4910803768049,-9.90655353511427));
#41963=CARTESIAN_POINT('Ctrl Pts',(-19.8196384388055,21.5310699717064,-9.91093999712681));
#41964=CARTESIAN_POINT('Ctrl Pts',(-19.7393618185147,21.5669561657756,-9.91532645913934));
#41965=CARTESIAN_POINT('Ctrl Pts',(-19.6576188802167,21.5985778865007,-9.91971292115187));
#41966=CARTESIAN_POINT('Ctrl Pts',(-19.5796370556819,21.6287446449807,-9.92389755554492));
#41967=CARTESIAN_POINT('Ctrl Pts',(-19.5000306196521,21.6551430224068,-9.92808218993797));
#41968=CARTESIAN_POINT('Ctrl Pts',(-19.4191985515815,21.6775974428168,-9.93226682433101));
#41969=CARTESIAN_POINT('Ctrl Pts',(-19.3384815379547,21.7000199021387,-9.93644550241496));
#41970=CARTESIAN_POINT('Ctrl Pts',(-19.2565427969408,21.7185094330108,-9.9406241804989));
#41971=CARTESIAN_POINT('Ctrl Pts',(-19.1738002903986,21.7329388780391,-9.94480285858285));
#41972=CARTESIAN_POINT('Ctrl Pts',(-19.0895746838927,21.7476269604994,-9.94905643646829));
#41973=CARTESIAN_POINT('Ctrl Pts',(-19.0045166631074,21.758107797425,-9.95331001435372));
#41974=CARTESIAN_POINT('Ctrl Pts',(-18.9190822179584,21.7643007211442,-9.95756359223916));
#41975=CARTESIAN_POINT('Ctrl Pts',(-18.8353040862403,21.7703735829526,-9.96173470621711));
#41976=CARTESIAN_POINT('Ctrl Pts',(-18.7511644753126,21.7723232722254,-9.96590582019506));
#41977=CARTESIAN_POINT('Ctrl Pts',(-18.6671008395073,21.7701257300737,-9.97007693417301));
#41978=CARTESIAN_POINT('Ctrl Pts',(-18.5830654120668,21.7679289253285,-9.97424664849338));
#41979=CARTESIAN_POINT('Ctrl Pts',(-18.49910636861,21.7615876649968,-9.97841636281376));
#41980=CARTESIAN_POINT('Ctrl Pts',(-18.4156612239222,21.7511300013277,-9.98258607713413));
#41981=CARTESIAN_POINT('Ctrl Pts',(-18.3322190485709,21.7406727097873,-9.98675564307817));
#41982=CARTESIAN_POINT('Ctrl Pts',(-18.2492911919861,21.7260993641991,-9.99092520902222));
#41983=CARTESIAN_POINT('Ctrl Pts',(-18.1673087413396,21.7074897390852,-9.99509477496626));
#41984=CARTESIAN_POINT('Ctrl Pts',(-18.0824438888646,21.6882258225098,-9.99941093770518));
#41985=CARTESIAN_POINT('Ctrl Pts',(-17.9985926745537,21.664636631037,-10.0037271004441));
#41986=CARTESIAN_POINT('Ctrl Pts',(-17.9162183607825,21.6368675129855,-10.008043263183));
#41987=CARTESIAN_POINT('Ctrl Pts',(-17.8365273816181,21.6100029710338,-10.0122188273747));
#41988=CARTESIAN_POINT('Ctrl Pts',(-17.7582189816852,21.5792268589617,-10.0163943915664));
#41989=CARTESIAN_POINT('Ctrl Pts',(-17.6816923706305,21.5447199174645,-10.0205699557581));
#41990=CARTESIAN_POINT('Ctrl Pts',(-17.6013005823761,21.5084701123848,-10.0249564177706));
#41991=CARTESIAN_POINT('Ctrl Pts',(-17.522875828849,21.4681029519009,-10.0293428797831));
#41992=CARTESIAN_POINT('Ctrl Pts',(-17.4468498189206,21.423881472503,-10.0337293417957));
#41993=CARTESIAN_POINT('Ctrl Pts',(-17.3708238089921,21.3796599931052,-10.0381158038082));
#41994=CARTESIAN_POINT('Ctrl Pts',(-17.2971969868963,21.3315845757053,-10.0425022658208));
#41995=CARTESIAN_POINT('Ctrl Pts',(-17.2263622218889,21.2799679383722,-10.0468887278333));
#41996=CARTESIAN_POINT('Ctrl Pts',(-17.2089081629896,21.2672493272763,-10.047969575159));
#41997=CARTESIAN_POINT('Ctrl Pts',(-17.19160669479,21.2543037392071,-10.0490504224848));
#41998=CARTESIAN_POINT('Ctrl Pts',(-17.1744642439897,21.2411350264762,-10.0501312698105));
#41999=CARTESIAN_POINT('Ctrl Pts',(-17.1744642439897,21.2411350264762,-9.25004023969326));
#42000=CARTESIAN_POINT('Ctrl Pts',(-17.1077984582143,21.1899228286354,-9.25421687978312));
#42001=CARTESIAN_POINT('Ctrl Pts',(-17.0437157308937,21.1354678945878,-9.25839351987297));
#42002=CARTESIAN_POINT('Ctrl Pts',(-16.9825323856757,21.0780728951953,-9.26257015996283));
#42003=CARTESIAN_POINT('Ctrl Pts',(-16.9212438722431,21.020579239386,-9.26675397929042));
#42004=CARTESIAN_POINT('Ctrl Pts',(-16.8628650136832,20.9601357565965,-9.27093779861802));
#42005=CARTESIAN_POINT('Ctrl Pts',(-16.8076738254214,20.8970805049384,-9.27512161794562));
#42006=CARTESIAN_POINT('Ctrl Pts',(-16.7693642901206,20.8533123335079,-9.27802570787865));
#42007=CARTESIAN_POINT('Ctrl Pts',(-16.7325897638593,20.8082865027903,-9.28092979781168));
#42008=CARTESIAN_POINT('Ctrl Pts',(-16.6974308899393,20.7621241923026,-9.28383388774471));
#42009=CARTESIAN_POINT('Ctrl Pts',(-16.6467688800087,20.6956068334797,-9.28801852213775));
#42010=CARTESIAN_POINT('Ctrl Pts',(-16.5992748500802,20.6264810343216,-9.2922031565308));
#42011=CARTESIAN_POINT('Ctrl Pts',(-16.5552283987658,20.5550812139358,-9.29638779092385));
#42012=CARTESIAN_POINT('Ctrl Pts',(-16.5112446421229,20.4837830223567,-9.30056646900779));
#42013=CARTESIAN_POINT('Ctrl Pts',(-16.470698956314,20.4102176270062,-9.30474514709174));
#42014=CARTESIAN_POINT('Ctrl Pts',(-16.4338297096936,20.3347511448678,-9.30892382517568));
#42015=CARTESIAN_POINT('Ctrl Pts',(-16.396299608325,20.2579319802739,-9.31317740306111));
#42016=CARTESIAN_POINT('Ctrl Pts',(-16.3625793350039,20.1791432881301,-9.31743098094655));
#42017=CARTESIAN_POINT('Ctrl Pts',(-16.3328731767862,20.0988006413847,-9.32168455883199));
#42018=CARTESIAN_POINT('Ctrl Pts',(-16.3037429304124,20.0200155936223,-9.32585567280994));
#42019=CARTESIAN_POINT('Ctrl Pts',(-16.2784727120492,19.9397367578111,-9.33002678678789));
#42020=CARTESIAN_POINT('Ctrl Pts',(-16.2572072783656,19.8583776440834,-9.33419790076584));
#42021=CARTESIAN_POINT('Ctrl Pts',(-16.2359489805037,19.777045831192,-9.33836761508621));
#42022=CARTESIAN_POINT('Ctrl Pts',(-16.2186929146628,19.6946349050203,-9.34253732940659));
#42023=CARTESIAN_POINT('Ctrl Pts',(-16.2055337985359,19.6115729247638,-9.34670704372696));
#42024=CARTESIAN_POINT('Ctrl Pts',(-16.1923751506669,19.528513900209,-9.350876609671));
#42025=CARTESIAN_POINT('Ctrl Pts',(-16.1833132337911,19.4448043221316,-9.35504617561504));
#42026=CARTESIAN_POINT('Ctrl Pts',(-16.1783912959603,19.3608804584879,-9.35921574155909));
#42027=CARTESIAN_POINT('Ctrl Pts',(-16.1732963088673,19.2740059353298,-9.36353190429801));
#42028=CARTESIAN_POINT('Ctrl Pts',(-16.1726378716504,19.1869023041989,-9.36784806703693));
#42029=CARTESIAN_POINT('Ctrl Pts',(-16.1764051921425,19.1000549738833,-9.37216422977585));
#42030=CARTESIAN_POINT('Ctrl Pts',(-16.1800497925657,19.016036686218,-9.37633979396753));
#42031=CARTESIAN_POINT('Ctrl Pts',(-16.1878361499306,18.9322587224488,-9.38051535815921));
#42032=CARTESIAN_POINT('Ctrl Pts',(-16.1997016639331,18.8491548068463,-9.38469092235089));
#42033=CARTESIAN_POINT('Ctrl Pts',(-16.2121664768403,18.7618535100274,-9.38907738436343));
#42034=CARTESIAN_POINT('Ctrl Pts',(-16.2291332400404,18.6752967161991,-9.39346384637597));
#42035=CARTESIAN_POINT('Ctrl Pts',(-16.2504693406595,18.5899722517347,-9.39785030838851));
#42036=CARTESIAN_POINT('Ctrl Pts',(-16.2718054412786,18.5046477872702,-9.40223677040106));
#42037=CARTESIAN_POINT('Ctrl Pts',(-16.2975106369606,18.4205561848056,-9.4066232324136));
#42038=CARTESIAN_POINT('Ctrl Pts',(-16.3273937923111,18.3381617783842,-9.41100969442614));
#42039=CARTESIAN_POINT('Ctrl Pts',(-16.3559019793865,18.2595584607401,-9.41519432881919));
#42040=CARTESIAN_POINT('Ctrl Pts',(-16.3883182194788,18.1822070136537,-9.41937896321224));
#42041=CARTESIAN_POINT('Ctrl Pts',(-16.4245126604673,18.1065235500301,-9.42356359760528));
#42042=CARTESIAN_POINT('Ctrl Pts',(-16.460655583149,18.0309478124493,-9.42774227568923));
#42043=CARTESIAN_POINT('Ctrl Pts',(-16.500565827944,17.9570357539527,-9.43192095377317));
#42044=CARTESIAN_POINT('Ctrl Pts',(-16.5440645726776,17.8851859767833,-9.43609963185711));
#42045=CARTESIAN_POINT('Ctrl Pts',(-16.5883430011486,17.8120483439956,-9.44035320974255));
#42046=CARTESIAN_POINT('Ctrl Pts',(-16.6363396782675,17.7410481057698,-9.44460678762798));
#42047=CARTESIAN_POINT('Ctrl Pts',(-16.6878157496594,17.6725819769457,-9.44886036551342));
#42048=CARTESIAN_POINT('Ctrl Pts',(-16.7382938569602,17.6054431976296,-9.45303147949137));
#42049=CARTESIAN_POINT('Ctrl Pts',(-16.7921173635638,17.5407415318688,-9.45720259346933));
#42050=CARTESIAN_POINT('Ctrl Pts',(-16.8490169269279,17.4788225223056,-9.46137370744728));
#42051=CARTESIAN_POINT('Ctrl Pts',(-16.905897397094,17.416924290264,-9.46554342176765));
#42052=CARTESIAN_POINT('Ctrl Pts',(-16.9658515630401,17.3578071984336,-9.46971313608802));
#42053=CARTESIAN_POINT('Ctrl Pts',(-17.0285707636154,17.3017825897283,-9.4738828504084));
#42054=CARTESIAN_POINT('Ctrl Pts',(-17.0912877323723,17.2457599746191,-9.47805241635244));
#42055=CARTESIAN_POINT('Ctrl Pts',(-17.1567691964755,17.1928299296704,-9.48222198229649));
#42056=CARTESIAN_POINT('Ctrl Pts',(-17.2246717329646,17.1432649632199,-9.48639154824053));
#42057=CARTESIAN_POINT('Ctrl Pts',(-17.2949616388698,17.0919573536941,-9.49070771097945));
#42058=CARTESIAN_POINT('Ctrl Pts',(-17.3678456086251,17.0442561687145,-9.49502387371837));
#42059=CARTESIAN_POINT('Ctrl Pts',(-17.442909648662,17.000415076347,-9.49934003645729));
#42060=CARTESIAN_POINT('Ctrl Pts',(-17.51552848549,16.9580021029521,-9.50351560064897));
#42061=CARTESIAN_POINT('Ctrl Pts',(-17.5901871024314,16.9192017744647,-9.50769116484065));
#42062=CARTESIAN_POINT('Ctrl Pts',(-17.6664869216557,16.8841962206572,-9.51186672903233));
#42063=CARTESIAN_POINT('Ctrl Pts',(-17.7466404633633,16.8474226195448,-9.51625319104487));
#42064=CARTESIAN_POINT('Ctrl Pts',(-17.8286048161833,16.8148374315278,-9.52063965305741));
#42065=CARTESIAN_POINT('Ctrl Pts',(-17.9118980145026,16.7865932013292,-9.52502611506995));
#42066=CARTESIAN_POINT('Ctrl Pts',(-17.9951912128219,16.7583489711306,-9.52941257708249));
#42067=CARTESIAN_POINT('Ctrl Pts',(-18.0798126775951,16.7344457832731,-9.53379903909503));
#42068=CARTESIAN_POINT('Ctrl Pts',(-18.1652685194102,16.7149742583487,-9.53818550110756));
#42069=CARTESIAN_POINT('Ctrl Pts',(-18.2467924112676,16.6963986471497,-9.54237013550061));
#42070=CARTESIAN_POINT('Ctrl Pts',(-18.3293790330748,16.6817867038644,-9.54655476989366));
#42071=CARTESIAN_POINT('Ctrl Pts',(-18.4126082132396,16.6712544774323,-9.55073940428671));
#42072=CARTESIAN_POINT('Ctrl Pts',(-18.4957189269681,16.6607372423208,-9.55491808237065));
#42073=CARTESIAN_POINT('Ctrl Pts',(-18.5794699298767,16.654288246849,-9.5590967604546));
#42074=CARTESIAN_POINT('Ctrl Pts',(-18.6634292675078,16.6519728857014,-9.56327543853854));
#42075=CARTESIAN_POINT('Ctrl Pts',(-18.7488935159254,16.6496160233692,-9.56752901642397));
#42076=CARTESIAN_POINT('Ctrl Pts',(-18.8345731712375,16.6515425508617,-9.57178259430941));
#42077=CARTESIAN_POINT('Ctrl Pts',(-18.9200053717024,16.6577663636679,-9.57603617219484));
#42078=CARTESIAN_POINT('Ctrl Pts',(-19.0037813022539,16.663869515718,-9.5802072861728));
#42079=CARTESIAN_POINT('Ctrl Pts',(-19.0873188071791,16.6741047825048,-9.58437840015075));
#42080=CARTESIAN_POINT('Ctrl Pts',(-19.1701815497895,16.6884327252533,-9.5885495141287));
#42081=CARTESIAN_POINT('Ctrl Pts',(-19.2530164870063,16.7027558601221,-9.59271922844908));
#42082=CARTESIAN_POINT('Ctrl Pts',(-19.335176658659,16.7211688651668,-9.59688894276945));
#42083=CARTESIAN_POINT('Ctrl Pts',(-19.4162332022013,16.7435807292205,-9.60105865708982));
#42084=CARTESIAN_POINT('Ctrl Pts',(-19.4972868614039,16.7659917957639,-9.60522822303387));
#42085=CARTESIAN_POINT('Ctrl Pts',(-19.5772365274094,16.7924013149753,-9.60939778897791));
#42086=CARTESIAN_POINT('Ctrl Pts',(-19.6556671754964,16.8226680260876,-9.61356735492195));
#42087=CARTESIAN_POINT('Ctrl Pts',(-19.7368553484154,16.8539988774245,-9.61788351766088));
#42088=CARTESIAN_POINT('Ctrl Pts',(-19.8164152065818,16.8894630151455,-9.6221996803998));
#42089=CARTESIAN_POINT('Ctrl Pts',(-19.8939093684294,16.9288496418882,-9.62651584313872));
#42090=CARTESIAN_POINT('Ctrl Pts',(-19.9688791661058,16.9669532534075,-9.6306914073304));
#42091=CARTESIAN_POINT('Ctrl Pts',(-20.0419153954163,17.0087274533691,-9.63486697152208));
#42092=CARTESIAN_POINT('Ctrl Pts',(-20.1126491714249,17.0539356842854,-9.63904253571376));
#42093=CARTESIAN_POINT('Ctrl Pts',(-20.1869555423062,17.1014272754729,-9.6434289977263));
#42094=CARTESIAN_POINT('Ctrl Pts',(-20.2587202783153,17.1527085808079,-9.64781545973884));
#42095=CARTESIAN_POINT('Ctrl Pts',(-20.3275542346358,17.2074569130477,-9.65220192175138));
#42096=CARTESIAN_POINT('Ctrl Pts',(-20.3963881909563,17.2622052452875,-9.65658838376392));
#42097=CARTESIAN_POINT('Ctrl Pts',(-20.4622909830917,17.3204201632972,-9.66097484577647));
#42098=CARTESIAN_POINT('Ctrl Pts',(-20.5249190804939,17.3817354354487,-9.66536130778901));
#42099=CARTESIAN_POINT('Ctrl Pts',(-20.5852113014986,17.440763796406,-9.66958416538902));
#42100=CARTESIAN_POINT('Ctrl Pts',(-20.6427127908696,17.5029045422552,-9.67380702298903));
#42101=CARTESIAN_POINT('Ctrl Pts',(-20.6970796830689,17.5678572314245,-9.67802988058905));
#42102=CARTESIAN_POINT('Ctrl Pts',(-20.7500936846377,17.6311936081461,-9.68214765466765));
#42103=CARTESIAN_POINT('Ctrl Pts',(-20.8001269202378,17.697203245602,-9.68626542874624));
#42104=CARTESIAN_POINT('Ctrl Pts',(-20.8468954124061,17.7655682388181,-9.69038320282484));
#42105=CARTESIAN_POINT('Ctrl Pts',(-20.89361966769,17.8338685676809,-9.69449708202705));
#42106=CARTESIAN_POINT('Ctrl Pts',(-20.9370850392269,17.9045194435154,-9.69861096122926));
#42107=CARTESIAN_POINT('Ctrl Pts',(-20.9770478427322,17.9771700379653,-9.70272484043147));
#42108=CARTESIAN_POINT('Ctrl Pts',(-21.016985643432,18.0497751784301,-9.70683614577719));
#42109=CARTESIAN_POINT('Ctrl Pts',(-21.0534249974544,18.1243771397533,-9.71094745112291));
#42110=CARTESIAN_POINT('Ctrl Pts',(-21.0861664418209,18.2005975900803,-9.71505875646863));
#42111=CARTESIAN_POINT('Ctrl Pts',(-21.1204445396303,18.2803952930204,-9.71936301761202));
#42112=CARTESIAN_POINT('Ctrl Pts',(-21.1506688210159,18.3619666588744,-9.72366727875541));
#42113=CARTESIAN_POINT('Ctrl Pts',(-21.1766659614561,18.4448518415192,-9.7279715398988));
#42114=CARTESIAN_POINT('Ctrl Pts',(-21.2014998963996,18.5240284432037,-9.73208321292915));
#42115=CARTESIAN_POINT('Ctrl Pts',(-21.2224767553181,18.6044033134951,-9.7361948859595));
#42116=CARTESIAN_POINT('Ctrl Pts',(-21.2394965458158,18.6855601281733,-9.74030655898986));
#42117=CARTESIAN_POINT('Ctrl Pts',(-21.2565208804897,18.7667386112071,-9.74441932981087));
#42118=CARTESIAN_POINT('Ctrl Pts',(-21.2695859645565,18.8486989864203,-9.74853210063189));
#42119=CARTESIAN_POINT('Ctrl Pts',(-21.2786432445869,18.9310165044542,-9.7526448714529));
#42120=CARTESIAN_POINT('Ctrl Pts',(-21.2877094512627,19.0134151527261,-9.75676169572553));
#42121=CARTESIAN_POINT('Ctrl Pts',(-21.2927599450141,19.0961711731438,-9.76087851999816));
#42122=CARTESIAN_POINT('Ctrl Pts',(-21.2937982075177,19.1788575547119,-9.76499534427079));
#42123=CARTESIAN_POINT('Ctrl Pts',(-21.2939423435977,19.1903364349236,-9.76556685957696));
#42124=CARTESIAN_POINT('Ctrl Pts',(-21.2940092371596,19.2018139780893,-9.76613837488313));
#42125=CARTESIAN_POINT('Ctrl Pts',(-21.2939989766127,19.2132890482674,-9.7667098901893));
#42126=CARTESIAN_POINT('Origin',(-18.734,19.211,1.76670989022852));
#42127=CARTESIAN_POINT('',(-17.1744642439897,21.2411350264762,-8.45013429617857));
#42128=CARTESIAN_POINT('',(-17.1744642439897,21.2411350264762,-8.51667714376075));
#42129=CARTESIAN_POINT('',(-17.1744642439897,21.2411350264762,1.76670989022852));
#42130=CARTESIAN_POINT('',(-21.2943302600992,19.210357489227,-9.03329016591285));
#42131=CARTESIAN_POINT('Ctrl Pts',(-17.1744642439897,21.2411350264762,-8.51667714376075));
#42132=CARTESIAN_POINT('Ctrl Pts',(-17.1602591749695,21.2302227902137,-8.51757292642982));
#42133=CARTESIAN_POINT('Ctrl Pts',(-17.1461740411721,21.2191656025168,-8.51846870909889));
#42134=CARTESIAN_POINT('Ctrl Pts',(-17.1322119090443,21.2079664272772,-8.51936449176795));
#42135=CARTESIAN_POINT('Ctrl Pts',(-17.0669880324057,21.1556496594946,-8.523549126161));
#42136=CARTESIAN_POINT('Ctrl Pts',(-17.0042085866861,21.1000367097147,-8.52773376055405));
#42137=CARTESIAN_POINT('Ctrl Pts',(-16.9442256444347,21.0413845924179,-8.5319183949471));
#42138=CARTESIAN_POINT('Ctrl Pts',(-16.8843280804773,20.9828159591504,-8.53609707303104));
#42139=CARTESIAN_POINT('Ctrl Pts',(-16.8272194396167,20.9212170697946,-8.54027575111498));
#42140=CARTESIAN_POINT('Ctrl Pts',(-16.7732194376018,20.8568856540237,-8.54445442919893));
#42141=CARTESIAN_POINT('Ctrl Pts',(-16.7182515243598,20.7914011438593,-8.54870800708436));
#42142=CARTESIAN_POINT('Ctrl Pts',(-16.6665051669309,20.723085484341,-8.5529615849698));
#42143=CARTESIAN_POINT('Ctrl Pts',(-16.6182789494494,20.6522926268656,-8.55721516285523));
#42144=CARTESIAN_POINT('Ctrl Pts',(-16.5709876912995,20.5828722270733,-8.56138627683319));
#42145=CARTESIAN_POINT('Ctrl Pts',(-16.527081572471,20.5110702205224,-8.56555739081114));
#42146=CARTESIAN_POINT('Ctrl Pts',(-16.4868009099954,20.4372529306315,-8.56972850478909));
#42147=CARTESIAN_POINT('Ctrl Pts',(-16.446533764085,20.3634604108451,-8.57389821910947));
#42148=CARTESIAN_POINT('Ctrl Pts',(-16.4098898786011,20.2876543542439,-8.57806793342984));
#42149=CARTESIAN_POINT('Ctrl Pts',(-16.3770645250476,20.2102272849111,-8.58223764775021));
#42150=CARTESIAN_POINT('Ctrl Pts',(-16.3442403395611,20.1328029707657,-8.58640721369426));
#42151=CARTESIAN_POINT('Ctrl Pts',(-16.3152345946181,20.0537581824513,-8.5905767796383));
#42152=CARTESIAN_POINT('Ctrl Pts',(-16.2901945969737,19.973505837446,-8.59474634558234));
#42153=CARTESIAN_POINT('Ctrl Pts',(-16.2642742239022,19.8904319189923,-8.59906250832126));
#42154=CARTESIAN_POINT('Ctrl Pts',(-16.2426038152404,19.8060644520148,-8.60337867106018));
#42155=CARTESIAN_POINT('Ctrl Pts',(-16.225290101654,19.7208770890525,-8.6076948337991));
#42156=CARTESIAN_POINT('Ctrl Pts',(-16.2085403804666,19.6384646954785,-8.61187039799078));
#42157=CARTESIAN_POINT('Ctrl Pts',(-16.1958678987932,19.5552854746203,-8.61604596218246));
#42158=CARTESIAN_POINT('Ctrl Pts',(-16.1873166326445,19.471775432959,-8.62022152637414));
#42159=CARTESIAN_POINT('Ctrl Pts',(-16.1783334623714,19.3840474976197,-8.62460798838669));
#42160=CARTESIAN_POINT('Ctrl Pts',(-16.173898803398,19.2959550268228,-8.62899445039922));
#42161=CARTESIAN_POINT('Ctrl Pts',(-16.1740017537922,19.2080034331647,-8.63338091241176));
#42162=CARTESIAN_POINT('Ctrl Pts',(-16.1741047041864,19.1200518395067,-8.63776737442431));
#42163=CARTESIAN_POINT('Ctrl Pts',(-16.1787451573697,19.0322416983818,-8.64215383643685));
#42164=CARTESIAN_POINT('Ctrl Pts',(-16.1878497481281,18.9450697555886,-8.64654029844939));
#42165=CARTESIAN_POINT('Ctrl Pts',(-16.1965354231695,18.8619087231031,-8.65072493284244));
#42166=CARTESIAN_POINT('Ctrl Pts',(-16.2093157897326,18.7790189093826,-8.65490956723549));
#42167=CARTESIAN_POINT('Ctrl Pts',(-16.2261653095063,18.6968354687883,-8.65909420162853));
#42168=CARTESIAN_POINT('Ctrl Pts',(-16.2429908460741,18.6147690061494,-8.66327287971248));
#42169=CARTESIAN_POINT('Ctrl Pts',(-16.2638739396399,18.5334073663311,-8.66745155779642));
#42170=CARTESIAN_POINT('Ctrl Pts',(-16.2887373027363,18.4531805351071,-8.67163023588037));
#42171=CARTESIAN_POINT('Ctrl Pts',(-16.3140463237472,18.3715156955915,-8.6758838137658));
#42172=CARTESIAN_POINT('Ctrl Pts',(-16.3434796603857,18.2910272272441,-8.68013739165124));
#42173=CARTESIAN_POINT('Ctrl Pts',(-16.3769013134697,18.2121577792479,-8.68439096953667));
#42174=CARTESIAN_POINT('Ctrl Pts',(-16.4096750225917,18.1348173694021,-8.68856208351463));
#42175=CARTESIAN_POINT('Ctrl Pts',(-16.4462835978107,18.0590342074479,-8.69273319749258));
#42176=CARTESIAN_POINT('Ctrl Pts',(-16.4865490981547,17.9852086458966,-8.69690431147053));
#42177=CARTESIAN_POINT('Ctrl Pts',(-16.5268010870212,17.9114078572255,-8.70107402579091));
#42178=CARTESIAN_POINT('Ctrl Pts',(-16.570707343848,17.8395637678914,-8.70524374011128));
#42179=CARTESIAN_POINT('Ctrl Pts',(-16.6180435147611,17.7700530361685,-8.70941345443165));
#42180=CARTESIAN_POINT('Ctrl Pts',(-16.6653780012501,17.7005447779356,-8.71358302037569));
#42181=CARTESIAN_POINT('Ctrl Pts',(-16.7161418995134,17.6333700919857,-8.71775258631974));
#42182=CARTESIAN_POINT('Ctrl Pts',(-16.7700677456501,17.5688763443869,-8.72192215226378));
#42183=CARTESIAN_POINT('Ctrl Pts',(-16.8258895580122,17.5021150761843,-8.72623831500271));
#42184=CARTESIAN_POINT('Ctrl Pts',(-16.8850994651023,17.4382271821969,-8.73055447774162));
#42185=CARTESIAN_POINT('Ctrl Pts',(-16.9473569713774,17.3775587851599,-8.73487064048054));
#42186=CARTESIAN_POINT('Ctrl Pts',(-17.007586445934,17.3188666547752,-8.73904620467222));
#42187=CARTESIAN_POINT('Ctrl Pts',(-17.0706676333014,17.2631877685198,-8.7432217688639));
#42188=CARTESIAN_POINT('Ctrl Pts',(-17.1362577244093,17.2107951052979,-8.74739733305558));
#42189=CARTESIAN_POINT('Ctrl Pts',(-17.2051606150934,17.1557562132084,-8.75178379506812));
#42190=CARTESIAN_POINT('Ctrl Pts',(-17.2768320453054,17.1043445831753,-8.75617025708067));
#42191=CARTESIAN_POINT('Ctrl Pts',(-17.3508411420262,17.0568246186514,-8.76055671909321));
#42192=CARTESIAN_POINT('Ctrl Pts',(-17.4248502387469,17.0093046541275,-8.76494318110575));
#42193=CARTESIAN_POINT('Ctrl Pts',(-17.5011964604717,16.9656765769471,-8.76932964311829));
#42194=CARTESIAN_POINT('Ctrl Pts',(-17.5794224113971,16.926147577655,-8.77371610513083));
#42195=CARTESIAN_POINT('Ctrl Pts',(-17.6540490703618,16.8884373662163,-8.77790073952388));
#42196=CARTESIAN_POINT('Ctrl Pts',(-17.730664056125,16.8543169479217,-8.78208537391692));
#42197=CARTESIAN_POINT('Ctrl Pts',(-17.8088876493305,16.8240003898956,-8.78627000830997));
#42198=CARTESIAN_POINT('Ctrl Pts',(-17.8869999009331,16.7937269837374,-8.79044868639391));
#42199=CARTESIAN_POINT('Ctrl Pts',(-17.9667157867297,16.7672468481169,-8.79462736447786));
#42200=CARTESIAN_POINT('Ctrl Pts',(-18.0476319224908,16.7447277396491,-8.7988060425618));
#42201=CARTESIAN_POINT('Ctrl Pts',(-18.1299984218321,16.7218049923463,-8.80305962044724));
#42202=CARTESIAN_POINT('Ctrl Pts',(-18.213608193011,16.7029868892008,-8.80731319833267));
#42203=CARTESIAN_POINT('Ctrl Pts',(-18.2980154243377,16.6883986740302,-8.81156677621811));
#42204=CARTESIAN_POINT('Ctrl Pts',(-18.380786256778,16.6740932798773,-8.81573789019606));
#42205=CARTESIAN_POINT('Ctrl Pts',(-18.4643234304655,16.6638553099794,-8.81990900417401));
#42206=CARTESIAN_POINT('Ctrl Pts',(-18.5481939962223,16.6577518473599,-8.82408011815197));
#42207=CARTESIAN_POINT('Ctrl Pts',(-18.6320364184008,16.6516504328163,-8.82824983247234));
#42208=CARTESIAN_POINT('Ctrl Pts',(-18.7162115520294,16.6496808035662,-8.83241954679271));
#42209=CARTESIAN_POINT('Ctrl Pts',(-18.8002812486104,16.6518581914863,-8.83658926111308));
#42210=CARTESIAN_POINT('Ctrl Pts',(-18.8843479536308,16.6540355019256,-8.84075882705713));
#42211=CARTESIAN_POINT('Ctrl Pts',(-18.9683087692067,16.660359523368,-8.84492839300117));
#42212=CARTESIAN_POINT('Ctrl Pts',(-19.0517268423097,16.6707933836643,-8.84909795894522));
#42213=CARTESIAN_POINT('Ctrl Pts',(-19.1380777919556,16.681594085617,-8.85341412168414));
#42214=CARTESIAN_POINT('Ctrl Pts',(-19.2238466000237,16.6967989420232,-8.85773028442306));
#42215=CARTESIAN_POINT('Ctrl Pts',(-19.3085579282895,16.7163089996876,-8.86204644716198));
#42216=CARTESIAN_POINT('Ctrl Pts',(-19.3905097939472,16.7351835192757,-8.86622201135366));
#42217=CARTESIAN_POINT('Ctrl Pts',(-19.4714715762059,16.758086889941,-8.87039757554534));
#42218=CARTESIAN_POINT('Ctrl Pts',(-19.551028186959,16.7848786218092,-8.87457313973702));
#42219=CARTESIAN_POINT('Ctrl Pts',(-19.6346030129933,16.8130235403628,-8.87895960174956));
#42220=CARTESIAN_POINT('Ctrl Pts',(-19.716626443602,16.8454597306831,-8.8833460637621));
#42221=CARTESIAN_POINT('Ctrl Pts',(-19.7966429339306,16.8819680133224,-8.88773252577464));
#42222=CARTESIAN_POINT('Ctrl Pts',(-19.8766594242591,16.9184762959617,-8.89211898778718));
#42223=CARTESIAN_POINT('Ctrl Pts',(-19.9546684946739,16.959056335675,-8.89650544979972));
#42224=CARTESIAN_POINT('Ctrl Pts',(-20.0302483510423,17.003435683288,-8.90089191181226));
#42225=CARTESIAN_POINT('Ctrl Pts',(-20.102350666183,17.0457730713314,-8.90507654620531));
#42226=CARTESIAN_POINT('Ctrl Pts',(-20.1725107769709,17.0917254144961,-8.90926118059836));
#42227=CARTESIAN_POINT('Ctrl Pts',(-20.240343151946,17.1410892993693,-8.91344581499141));
#42228=CARTESIAN_POINT('Ctrl Pts',(-20.3080789759311,17.1903829208624,-8.91762449307535));
#42229=CARTESIAN_POINT('Ctrl Pts',(-20.373493276466,17.243078170329,-8.9218031711593));
#42230=CARTESIAN_POINT('Ctrl Pts',(-20.4362266525528,17.2989266689431,-8.92598184924324));
#42231=CARTESIAN_POINT('Ctrl Pts',(-20.5000844793203,17.3557762117573,-8.93023542712868));
#42232=CARTESIAN_POINT('Ctrl Pts',(-20.5611639093906,17.4158929154665,-8.93448900501411));
#42233=CARTESIAN_POINT('Ctrl Pts',(-20.6191183231213,17.4789697150938,-8.93874258289955));
#42234=CARTESIAN_POINT('Ctrl Pts',(-20.6759491774531,17.5408236478761,-8.9429136968775));
#42235=CARTESIAN_POINT('Ctrl Pts',(-20.7297747776526,17.6055235719756,-8.94708481085545));
#42236=CARTESIAN_POINT('Ctrl Pts',(-20.7803043703348,17.6727417564177,-8.9512559248334));
#42237=CARTESIAN_POINT('Ctrl Pts',(-20.8308170073241,17.7399373851488,-8.95542563915377));
#42238=CARTESIAN_POINT('Ctrl Pts',(-20.8780355571482,17.8096492285708,-8.95959535347414));
#42239=CARTESIAN_POINT('Ctrl Pts',(-20.9217100507379,17.8815171178612,-8.96376506779451));
#42240=CARTESIAN_POINT('Ctrl Pts',(-20.9653829902017,17.9533824497836,-8.96793463373855));
#42241=CARTESIAN_POINT('Ctrl Pts',(-21.0055118859952,18.0274032814579,-8.9721041996826));
#42242=CARTESIAN_POINT('Ctrl Pts',(-21.0418912815019,18.1031923304257,-8.97627376562664));
#42243=CARTESIAN_POINT('Ctrl Pts',(-21.0795497316758,18.1816460288594,-8.98058992836556));
#42244=CARTESIAN_POINT('Ctrl Pts',(-21.1131898827321,18.2619941236263,-8.98490609110448));
#42245=CARTESIAN_POINT('Ctrl Pts',(-21.1426376470828,18.3437833690158,-8.9892222538434));
#42246=CARTESIAN_POINT('Ctrl Pts',(-21.171126153607,18.4229083383394,-8.99339781803508));
#42247=CARTESIAN_POINT('Ctrl Pts',(-21.1956911205896,18.5033815448835,-8.99757338222676));
#42248=CARTESIAN_POINT('Ctrl Pts',(-21.2162259984621,18.5847779207351,-9.00174894641844));
#42249=CARTESIAN_POINT('Ctrl Pts',(-21.2377980441989,18.6702854340294,-9.00613540843098));
#42250=CARTESIAN_POINT('Ctrl Pts',(-21.254922068569,18.7568112533014,-9.01052187044352));
#42251=CARTESIAN_POINT('Ctrl Pts',(-21.2675357890124,18.8438536997419,-9.01490833245606));
#42252=CARTESIAN_POINT('Ctrl Pts',(-21.2801495094559,18.9308961461825,-9.01929479446861));
#42253=CARTESIAN_POINT('Ctrl Pts',(-21.288252948244,19.0184546350337,-9.02368125648114));
#42254=CARTESIAN_POINT('Ctrl Pts',(-21.2918468828523,19.10602703261,-9.02806771849369));
#42255=CARTESIAN_POINT('Ctrl Pts',(-21.2932731600888,19.1407807303868,-9.02980851558629));
#42256=CARTESIAN_POINT('Ctrl Pts',(-21.2939911726516,19.1755636940745,-9.0315493126789));
#42257=CARTESIAN_POINT('Ctrl Pts',(-21.2939999191096,19.2103564484228,-9.0332901097715));
#42258=CARTESIAN_POINT('Ctrl Pts',(-21.2980344970333,19.2103691601534,-9.03329079544681));
#42259=CARTESIAN_POINT('Ctrl Pts',(-21.2952860334465,20.0241271385548,-9.07394170535625));
#42260=CARTESIAN_POINT('Ctrl Pts',(-20.4360629396139,21.691476034616,-9.15698455082618));
#42261=CARTESIAN_POINT('Ctrl Pts',(-18.2953377909523,21.9356233336023,-9.25149015500852));
#42262=CARTESIAN_POINT('Ctrl Pts',(-17.3565755020692,21.3826576096171,-9.30534484928144));
#42263=CARTESIAN_POINT('Ctrl Pts',(-17.1750494706848,21.2403917593382,-9.31680760799388));
#42264=CARTESIAN_POINT('',(-21.293999998394,19.2110906788005,-8.96670989026365));
#42265=CARTESIAN_POINT('Ctrl Pts',(-21.293999998394,19.2110906788005,-8.96670989026365));
#42266=CARTESIAN_POINT('Ctrl Pts',(-21.2939968622716,19.2996281672638,-8.97108917708311));
#42267=CARTESIAN_POINT('Ctrl Pts',(-21.2893963356695,19.3880718027693,-8.97546846390256));
#42268=CARTESIAN_POINT('Ctrl Pts',(-21.2802532223815,19.4759424985004,-8.97984775072202));
#42269=CARTESIAN_POINT('Ctrl Pts',(-21.2710840473103,19.5640636632957,-8.98423952038189));
#42270=CARTESIAN_POINT('Ctrl Pts',(-21.2573464424813,19.6516082364874,-8.98863129004176));
#42271=CARTESIAN_POINT('Ctrl Pts',(-21.2391468026208,19.7381048257401,-8.99302305970162));
#42272=CARTESIAN_POINT('Ctrl Pts',(-21.2209205771356,19.824727767266,-8.99742124475988));
#42273=CARTESIAN_POINT('Ctrl Pts',(-21.1982194166657,19.9102992971048,-9.00181942981815));
#42274=CARTESIAN_POINT('Ctrl Pts',(-21.1711995861977,19.9943633748381,-9.00621761487641));
#42275=CARTESIAN_POINT('Ctrl Pts',(-21.1441046030879,20.0786612674182,-9.01062803299537));
#42276=CARTESIAN_POINT('Ctrl Pts',(-21.1126670698914,20.1614429605725,-9.01503845111432));
#42277=CARTESIAN_POINT('Ctrl Pts',(-21.0770917883153,20.2422714829421,-9.01944886923327));
#42278=CARTESIAN_POINT('Ctrl Pts',(-21.0501146625114,20.3035646370618,-9.02279333761612));
#42279=CARTESIAN_POINT('Ctrl Pts',(-21.0207591774505,20.3637350853212,-9.02613780599898));
#42280=CARTESIAN_POINT('Ctrl Pts',(-20.989131617054,20.4226028184861,-9.02948227438183));
#42281=CARTESIAN_POINT('Ctrl Pts',(-20.9495588772781,20.4962587519987,-9.03366690877488));
#42282=CARTESIAN_POINT('Ctrl Pts',(-20.9063001320242,20.5681109610611,-9.03785154316793));
#42283=CARTESIAN_POINT('Ctrl Pts',(-20.8595440286337,20.6377664778581,-9.04203617756098));
#42284=CARTESIAN_POINT('Ctrl Pts',(-20.8128544767691,20.7073228486487,-9.04621485564492));
#42285=CARTESIAN_POINT('Ctrl Pts',(-20.7626777089519,20.7746883591287,-9.05039353372887));
#42286=CARTESIAN_POINT('Ctrl Pts',(-20.7092482964899,20.8394944480144,-9.05457221181281));
#42287=CARTESIAN_POINT('Ctrl Pts',(-20.6548612002085,20.9054621394682,-9.05882578969825));
#42288=CARTESIAN_POINT('Ctrl Pts',(-20.5971039332158,20.9687773268414,-9.06307936758368));
#42289=CARTESIAN_POINT('Ctrl Pts',(-20.5362701954423,21.0290819955712,-9.06733294546912));
#42290=CARTESIAN_POINT('Ctrl Pts',(-20.4766158383829,21.0882175406228,-9.07150405944707));
#42291=CARTESIAN_POINT('Ctrl Pts',(-20.4140035745829,21.1444579161298,-9.07567517342502));
#42292=CARTESIAN_POINT('Ctrl Pts',(-20.3487498736145,21.1975001499275,-9.07984628740297));
#42293=CARTESIAN_POINT('Ctrl Pts',(-20.2835180691557,21.2505245848913,-9.08401600172335));
#42294=CARTESIAN_POINT('Ctrl Pts',(-20.2156469445307,21.3003527195436,-9.08818571604372));
#42295=CARTESIAN_POINT('Ctrl Pts',(-20.1454869304126,21.3467211066228,-9.09235543036409));
#42296=CARTESIAN_POINT('Ctrl Pts',(-20.0753294128889,21.3930878437159,-9.09652499630814));
#42297=CARTESIAN_POINT('Ctrl Pts',(-20.0028835520724,21.4359948250818,-9.10069456225219));
#42298=CARTESIAN_POINT('Ctrl Pts',(-19.9285285607301,21.475222055718,-9.10486412819624));
#42299=CARTESIAN_POINT('Ctrl Pts',(-19.8515593396191,21.5158284673914,-9.10918029093516));
#42300=CARTESIAN_POINT('Ctrl Pts',(-19.7725447065604,21.5524913076845,-9.11349645367408));
#42301=CARTESIAN_POINT('Ctrl Pts',(-19.6919309796755,21.585019426664,-9.11781261641299));
#42302=CARTESIAN_POINT('Ctrl Pts',(-19.6139432364647,21.6164879455891,-9.12198818060467));
#42303=CARTESIAN_POINT('Ctrl Pts',(-19.5344594409715,21.6440868736177,-9.12616374479635));
#42304=CARTESIAN_POINT('Ctrl Pts',(-19.4539003149003,21.6676936187906,-9.13033930898803));
#42305=CARTESIAN_POINT('Ctrl Pts',(-19.3692723388824,21.6924926845425,-9.13472577100057));
#42306=CARTESIAN_POINT('Ctrl Pts',(-19.2834581156084,21.7128855434687,-9.13911223301311));
#42307=CARTESIAN_POINT('Ctrl Pts',(-19.1969566012277,21.7287909336122,-9.14349869502565));
#42308=CARTESIAN_POINT('Ctrl Pts',(-19.110455086847,21.7446963237556,-9.14788515703818));
#42309=CARTESIAN_POINT('Ctrl Pts',(-19.0232668665414,21.756114245197,-9.15227161905073));
#42310=CARTESIAN_POINT('Ctrl Pts',(-18.9358937423135,21.7630264334083,-9.15665808106326));
#42311=CARTESIAN_POINT('Ctrl Pts',(-18.8525619577015,21.7696189066009,-9.16084165250892));
#42312=CARTESIAN_POINT('Ctrl Pts',(-18.7687518984978,21.7721377831229,-9.16502522395457));
#42313=CARTESIAN_POINT('Ctrl Pts',(-18.6848957690166,21.7705290141937,-9.16920879540023));
#42314=CARTESIAN_POINT('Ctrl Pts',(-18.6011496143914,21.7689223551178,-9.17338688021455));
#42315=CARTESIAN_POINT('Ctrl Pts',(-18.5173579649434,21.7631988058255,-9.17756496502888));
#42316=CARTESIAN_POINT('Ctrl Pts',(-18.4339575044883,21.7533560924636,-9.18174304984321));
#42317=CARTESIAN_POINT('Ctrl Pts',(-18.3506413936366,21.7435233338307,-9.18591690902382));
#42318=CARTESIAN_POINT('Ctrl Pts',(-18.267716140326,21.7295797379285,-9.19009076820444));
#42319=CARTESIAN_POINT('Ctrl Pts',(-18.1856164183454,21.711575023344,-9.19426462738505));
#42320=CARTESIAN_POINT('Ctrl Pts',(-18.1035750976559,21.6935831163372,-9.19843551750853));
#42321=CARTESIAN_POINT('Ctrl Pts',(-18.0223585895858,21.6715359284619,-9.20260640763201));
#42322=CARTESIAN_POINT('Ctrl Pts',(-17.9423930915371,21.645534555613,-9.2067772977555));
#42323=CARTESIAN_POINT('Ctrl Pts',(-17.8624446940832,21.6195387431489,-9.21094729593553));
#42324=CARTESIAN_POINT('Ctrl Pts',(-17.7837472149607,21.5895905593654,-9.21511729411556));
#42325=CARTESIAN_POINT('Ctrl Pts',(-17.7067122821135,21.5558411342092,-9.21928729229559));
#42326=CARTESIAN_POINT('Ctrl Pts',(-17.6296873849862,21.5220961057568,-9.22345674722944));
#42327=CARTESIAN_POINT('Ctrl Pts',(-17.5543250225427,21.4845510104642,-9.22762620216328));
#42328=CARTESIAN_POINT('Ctrl Pts',(-17.4810158732245,21.4434047074956,-9.23179565709713));
#42329=CARTESIAN_POINT('Ctrl Pts',(-17.407668031838,21.4022366877893,-9.23596731264082));
#42330=CARTESIAN_POINT('Ctrl Pts',(-17.3363759656959,21.357463895993,-9.24013896818451));
#42331=CARTESIAN_POINT('Ctrl Pts',(-17.2675040274966,21.3093301843683,-9.2443106237282));
#42332=CARTESIAN_POINT('Ctrl Pts',(-17.2359730000249,21.28729355489,-9.24622049571655));
#42333=CARTESIAN_POINT('Ctrl Pts',(-17.204948823483,21.264553070649,-9.24813036770491));
#42334=CARTESIAN_POINT('Ctrl Pts',(-17.1744642439897,21.2411350264762,-9.25004023969326));
#42335=CARTESIAN_POINT('Ctrl Pts',(-17.1744642439897,21.2411350264762,-8.45013429617857));
#42336=CARTESIAN_POINT('Ctrl Pts',(-17.1077840465769,21.1899117577148,-8.45430378103253));
#42337=CARTESIAN_POINT('Ctrl Pts',(-17.0436167203881,21.1353895379119,-8.4584732658865));
#42338=CARTESIAN_POINT('Ctrl Pts',(-16.9822967584395,21.0778518295533,-8.46264275074046));
#42339=CARTESIAN_POINT('Ctrl Pts',(-16.9209699105371,21.0203076599707,-8.46681270380869));
#42340=CARTESIAN_POINT('Ctrl Pts',(-16.8624913963391,20.9597476451823,-8.47098265687691));
#42341=CARTESIAN_POINT('Ctrl Pts',(-16.807159597991,20.8964928256109,-8.47515260994513));
#42342=CARTESIAN_POINT('Ctrl Pts',(-16.7517686933345,20.8331704362336,-8.47932701742364));
#42343=CARTESIAN_POINT('Ctrl Pts',(-16.6995315186948,20.7671478420157,-8.48350142490214));
#42344=CARTESIAN_POINT('Ctrl Pts',(-16.6507064613291,20.6987795642272,-8.48767583238065));
#42345=CARTESIAN_POINT('Ctrl Pts',(-16.6018534047597,20.6303720799852,-8.49185263371371));
#42346=CARTESIAN_POINT('Ctrl Pts',(-16.5564166096692,20.5596166212149,-8.49602943504676));
#42347=CARTESIAN_POINT('Ctrl Pts',(-16.5146100453367,20.4868950697998,-8.50020623637982));
#42348=CARTESIAN_POINT('Ctrl Pts',(-16.4727323283785,20.4140497500386,-8.50439014641426));
#42349=CARTESIAN_POINT('Ctrl Pts',(-16.4344973889752,20.3392320654702,-8.50857405644871));
#42350=CARTESIAN_POINT('Ctrl Pts',(-16.4000721978852,20.2628464785868,-8.51275796648315));
#42351=CARTESIAN_POINT('Ctrl Pts',(-16.3780730591327,20.2140328897197,-8.51543166020746));
#42352=CARTESIAN_POINT('Ctrl Pts',(-16.3576287426084,20.1645794072701,-8.51810535393178));
#42353=CARTESIAN_POINT('Ctrl Pts',(-16.3387721302028,20.1145947386671,-8.52077904765609));
#42354=CARTESIAN_POINT('Ctrl Pts',(-16.3092593897977,20.0363630543649,-8.52496368204914));
#42355=CARTESIAN_POINT('Ctrl Pts',(-16.2835285016034,19.95653836908,-8.52914831644219));
#42356=CARTESIAN_POINT('Ctrl Pts',(-16.2617516946766,19.8755211184194,-8.53333295083524));
#42357=CARTESIAN_POINT('Ctrl Pts',(-16.2400058843389,19.7946191857871,-8.53751162891919));
#42358=CARTESIAN_POINT('Ctrl Pts',(-16.2222030943945,19.7125284999512,-8.54169030700313));
#42359=CARTESIAN_POINT('Ctrl Pts',(-16.2084669780844,19.6296680728378,-8.54586898508708));
#42360=CARTESIAN_POINT('Ctrl Pts',(-16.1944846517614,19.5453224321191,-8.55012256297252));
#42361=CARTESIAN_POINT('Ctrl Pts',(-16.1847163934876,19.4601796345795,-8.55437614085795));
#42362=CARTESIAN_POINT('Ctrl Pts',(-16.179239049994,19.3746963295992,-8.55862971874339));
#42363=CARTESIAN_POINT('Ctrl Pts',(-16.1738678954921,19.2908702852928,-8.56280083272134));
#42364=CARTESIAN_POINT('Ctrl Pts',(-16.1726227957354,19.2067172987628,-8.5669719466993));
#42365=CARTESIAN_POINT('Ctrl Pts',(-16.1755241458591,19.1226750104564,-8.57114306067725));
#42366=CARTESIAN_POINT('Ctrl Pts',(-16.1784245224067,19.0386609233514,-8.57531277499763));
#42367=CARTESIAN_POINT('Ctrl Pts',(-16.1854685696706,18.9547579200742,-8.579482489318));
#42368=CARTESIAN_POINT('Ctrl Pts',(-16.1966245729686,18.8714032651844,-8.58365220363838));
#42369=CARTESIAN_POINT('Ctrl Pts',(-16.2077801792882,18.7880515764109,-8.58782176958242));
#42370=CARTESIAN_POINT('Ctrl Pts',(-16.2230473888477,18.705248653083,-8.59199133552647));
#42371=CARTESIAN_POINT('Ctrl Pts',(-16.2423428203254,18.6234248992887,-8.59616090147052));
#42372=CARTESIAN_POINT('Ctrl Pts',(-16.2623166553703,18.5387243232516,-8.60047706420944));
#42373=CARTESIAN_POINT('Ctrl Pts',(-16.2866071262492,18.4550735664097,-8.60479322694835));
#42374=CARTESIAN_POINT('Ctrl Pts',(-16.3150650107316,18.372934657862,-8.60910938968727));
#42375=CARTESIAN_POINT('Ctrl Pts',(-16.3425958826202,18.2934714156207,-8.61328495387895));
#42376=CARTESIAN_POINT('Ctrl Pts',(-16.3740266108365,18.2154234566588,-8.61746051807063));
#42377=CARTESIAN_POINT('Ctrl Pts',(-16.4091731183431,18.1391884632431,-8.62163608226231));
#42378=CARTESIAN_POINT('Ctrl Pts',(-16.4460947923909,18.0591030215414,-8.62602254427484));
#42379=CARTESIAN_POINT('Ctrl Pts',(-16.48711720705,17.9810190212158,-8.63040900628739));
#42380=CARTESIAN_POINT('Ctrl Pts',(-16.5319737202491,17.9053659535359,-8.63479546829992));
#42381=CARTESIAN_POINT('Ctrl Pts',(-16.5768302334482,17.829712885856,-8.63918193031246));
#42382=CARTESIAN_POINT('Ctrl Pts',(-16.625520460569,17.7564911918506,-8.643568392325));
#42383=CARTESIAN_POINT('Ctrl Pts',(-16.677728404917,17.6860911085397,-8.64795485433754));
#42384=CARTESIAN_POINT('Ctrl Pts',(-16.7275341843548,17.6189302374198,-8.65213948873059));
#42385=CARTESIAN_POINT('Ctrl Pts',(-16.7807264703944,17.5540870443,-8.65632412312364));
#42386=CARTESIAN_POINT('Ctrl Pts',(-16.8370617843824,17.49192309476,-8.66050875751669));
#42387=CARTESIAN_POINT('Ctrl Pts',(-16.8933169120239,17.4298476279078,-8.66468743560064));
#42388=CARTESIAN_POINT('Ctrl Pts',(-16.952705875139,17.3704441676471,-8.66886611368458));
#42389=CARTESIAN_POINT('Ctrl Pts',(-17.014943282162,17.3140434899935,-8.67304479176854));
#42390=CARTESIAN_POINT('Ctrl Pts',(-17.0782962499765,17.2566318707276,-8.67729836965397));
#42391=CARTESIAN_POINT('Ctrl Pts',(-17.1446004956336,17.2023321299324,-8.68155194753941));
#42392=CARTESIAN_POINT('Ctrl Pts',(-17.2135136449486,17.151456059196,-8.68580552542484));
#42393=CARTESIAN_POINT('Ctrl Pts',(-17.2810907783913,17.1015663203672,-8.6899766394028));
#42394=CARTESIAN_POINT('Ctrl Pts',(-17.3511761736811,17.054968972992,-8.69414775338075));
#42395=CARTESIAN_POINT('Ctrl Pts',(-17.4234128839599,17.0119180526253,-8.6983188673587));
#42396=CARTESIAN_POINT('Ctrl Pts',(-17.4956253545128,16.9688815784106,-8.70248858167908));
#42397=CARTESIAN_POINT('Ctrl Pts',(-17.5699873115138,16.9293894030873,-8.70665829599945));
#42398=CARTESIAN_POINT('Ctrl Pts',(-17.6461139181108,16.8936515426394,-8.71082801031982));
#42399=CARTESIAN_POINT('Ctrl Pts',(-17.7222378157965,16.8579149538979,-8.71499757626387));
#42400=CARTESIAN_POINT('Ctrl Pts',(-17.8001258214376,16.8259326091334,-8.71916714220791));
#42401=CARTESIAN_POINT('Ctrl Pts',(-17.8793709005808,16.7978673674193,-8.72333670815196));
#42402=CARTESIAN_POINT('Ctrl Pts',(-17.9614021389473,16.7688153864287,-8.72765287089087));
#42403=CARTESIAN_POINT('Ctrl Pts',(-18.0448871586136,16.7439612602711,-8.73196903362979));
#42404=CARTESIAN_POINT('Ctrl Pts',(-18.129356695062,16.7234296042537,-8.73628519636871));
#42405=CARTESIAN_POINT('Ctrl Pts',(-18.2110746452452,16.7035667647714,-8.74046076056039));
#42406=CARTESIAN_POINT('Ctrl Pts',(-18.2937134844275,16.6877491532913,-8.74463632475206));
#42407=CARTESIAN_POINT('Ctrl Pts',(-18.3768391873479,16.676037248024,-8.74881188894374));
#42408=CARTESIAN_POINT('Ctrl Pts',(-18.4641633719102,16.6637338022641,-8.75319835095628));
#42409=CARTESIAN_POINT('Ctrl Pts',(-18.5520243141264,16.6559617726585,-8.75758481296882));
#42410=CARTESIAN_POINT('Ctrl Pts',(-18.6399165515113,16.6527294309005,-8.76197127498136));
#42411=CARTESIAN_POINT('Ctrl Pts',(-18.7278087888962,16.6494970891426,-8.76635773699389));
#42412=CARTESIAN_POINT('Ctrl Pts',(-18.8157317424278,16.65080435055,-8.77074419900643));
#42413=CARTESIAN_POINT('Ctrl Pts',(-18.903186241511,16.6565967398073,-8.77513066101897));
#42414=CARTESIAN_POINT('Ctrl Pts',(-18.9866168294529,16.6621226126484,-8.77931529541202));
#42415=CARTESIAN_POINT('Ctrl Pts',(-19.0699316687706,16.6717505167586,-8.78349992980506));
#42416=CARTESIAN_POINT('Ctrl Pts',(-19.1526949496533,16.6854714337124,-8.78768456419811));
#42417=CARTESIAN_POINT('Ctrl Pts',(-19.2353404272495,16.6991728206391,-8.79186324228204));
#42418=CARTESIAN_POINT('Ctrl Pts',(-19.3174354558604,16.7169555737482,-8.79604192036597));
#42419=CARTESIAN_POINT('Ctrl Pts',(-19.3985474281617,16.7387587666808,-8.8002205984499));
#42420=CARTESIAN_POINT('Ctrl Pts',(-19.4811132742726,16.7609527661771,-8.80447417633534));
#42421=CARTESIAN_POINT('Ctrl Pts',(-19.5626599937758,16.7873127240839,-8.80872775422078));
#42422=CARTESIAN_POINT('Ctrl Pts',(-19.6427400986355,16.8177195247669,-8.81298133210622));
#42423=CARTESIAN_POINT('Ctrl Pts',(-19.721267694399,16.8475368302847,-8.81715244608417));
#42424=CARTESIAN_POINT('Ctrl Pts',(-19.7983845845472,16.8812452961235,-8.82132356006213));
#42425=CARTESIAN_POINT('Ctrl Pts',(-19.8736839568162,16.9186822910915,-8.82549467404008));
#42426=CARTESIAN_POINT('Ctrl Pts',(-19.9489580616535,16.9561067237141,-8.82966438836045));
#42427=CARTESIAN_POINT('Ctrl Pts',(-20.0224154482667,16.9972569960429,-8.83383410268082));
#42428=CARTESIAN_POINT('Ctrl Pts',(-20.0936712215601,17.0419231988559,-8.83800381700119));
#42429=CARTESIAN_POINT('Ctrl Pts',(-20.1649244592672,17.0865878122538,-8.84217338294524));
#42430=CARTESIAN_POINT('Ctrl Pts',(-20.2339758500889,17.1347678623259,-8.84634294888928));
#42431=CARTESIAN_POINT('Ctrl Pts',(-20.3004681352881,17.1862092500392,-8.85051251483332));
#42432=CARTESIAN_POINT('Ctrl Pts',(-20.3692982072079,17.2394592534847,-8.85482867757224));
#42433=CARTESIAN_POINT('Ctrl Pts',(-20.4353854517826,17.29620387614,-8.85914484031116));
#42434=CARTESIAN_POINT('Ctrl Pts',(-20.4983710832764,17.3561159927106,-8.86346100305009));
#42435=CARTESIAN_POINT('Ctrl Pts',(-20.5593049644492,17.4140764783855,-8.86763656724176));
#42436=CARTESIAN_POINT('Ctrl Pts',(-20.6173359087924,17.4750008911684,-8.87181213143344));
#42437=CARTESIAN_POINT('Ctrl Pts',(-20.6721781340603,17.5385570202095,-8.87598769562512));
#42438=CARTESIAN_POINT('Ctrl Pts',(-20.7297903097515,17.6053232182381,-8.88037415763766));
#42439=CARTESIAN_POINT('Ctrl Pts',(-20.7838828183066,17.6749935141292,-8.88476061965021));
#42440=CARTESIAN_POINT('Ctrl Pts',(-20.8341751072843,17.7471473712345,-8.88914708166276));
#42441=CARTESIAN_POINT('Ctrl Pts',(-20.8844673962619,17.8193012283399,-8.8935335436753));
#42442=CARTESIAN_POINT('Ctrl Pts',(-20.930959223453,17.8939381139566,-8.89792000568785));
#42443=CARTESIAN_POINT('Ctrl Pts',(-20.9734262024012,17.9706088181549,-8.9023064677004));
#42444=CARTESIAN_POINT('Ctrl Pts',(-21.0159038253685,18.047298739271,-8.90669402914565));
#42445=CARTESIAN_POINT('Ctrl Pts',(-21.054500797719,18.1262856298352,-8.91108159059091));
#42446=CARTESIAN_POINT('Ctrl Pts',(-21.0889748257326,18.2071605854691,-8.91546915203617));
#42447=CARTESIAN_POINT('Ctrl Pts',(-21.1233545067053,18.2878142059939,-8.91984470579149));
#42448=CARTESIAN_POINT('Ctrl Pts',(-21.1536335666927,18.3703452363822,-8.92422025954681));
#42449=CARTESIAN_POINT('Ctrl Pts',(-21.1796158858341,18.4543211123894,-8.92859581330213));
#42450=CARTESIAN_POINT('Ctrl Pts',(-21.2055560013422,18.5381605845955,-8.93296425975244));
#42451=CARTESIAN_POINT('Ctrl Pts',(-21.2272131436812,18.6234398583861,-8.93733270620275));
#42452=CARTESIAN_POINT('Ctrl Pts',(-21.2444392039475,18.7097066694204,-8.94170115265306));
#42453=CARTESIAN_POINT('Ctrl Pts',(-21.2616295048393,18.7957944002037,-8.94606053069714));
#42454=CARTESIAN_POINT('Ctrl Pts',(-21.274406969619,18.8828651985172,-8.95041990874123));
#42455=CARTESIAN_POINT('Ctrl Pts',(-21.2826736357252,18.9704533339265,-8.95477928678531));
#42456=CARTESIAN_POINT('Ctrl Pts',(-21.2902149496553,19.0503561166423,-8.95875615459971));
#42457=CARTESIAN_POINT('Ctrl Pts',(-21.2940028463113,19.1306890276033,-8.96273302241411));
#42458=CARTESIAN_POINT('Ctrl Pts',(-21.293999998394,19.2110906780901,-8.96670989022851));
#42459=CARTESIAN_POINT('Origin',(-18.734,19.211,1.76670989022852));
#42460=CARTESIAN_POINT('',(-17.1732300852521,21.2427130357989,-7.65021347737831));
#42461=CARTESIAN_POINT('',(-17.1756294998725,21.2395871765567,-7.71658756787471));
#42462=CARTESIAN_POINT('',(-17.1744642439897,21.2411350264762,1.76670989022852));
#42463=CARTESIAN_POINT('',(-21.2939989173812,19.2133543591349,-8.2332901225083));
#42464=CARTESIAN_POINT('Ctrl Pts',(-17.1756294998728,21.2395871765569,-7.7165875678747));
#42465=CARTESIAN_POINT('Ctrl Pts',(-16.9627571463261,21.0789787236254,-7.72982826247625));
#42466=CARTESIAN_POINT('Ctrl Pts',(-16.1737485052776,20.2707708752208,-7.78546089263828));
#42467=CARTESIAN_POINT('Ctrl Pts',(-15.9391113864609,18.0482922133962,-7.88348545836079));
#42468=CARTESIAN_POINT('Ctrl Pts',(-18.1988330487837,16.2315893043347,-8.01066126504222));
#42469=CARTESIAN_POINT('Ctrl Pts',(-20.7208250384235,17.0720883649514,-8.12726281551246));
#42470=CARTESIAN_POINT('Ctrl Pts',(-21.28776986438,18.5735386239974,-8.20147243042222));
#42471=CARTESIAN_POINT('Ctrl Pts',(-21.2935817164968,19.2133537193276,-8.23329010977151));
#42472=CARTESIAN_POINT('Ctrl Pts',(-21.2939989173812,19.2133543591349,-8.2332901225083));
#42473=CARTESIAN_POINT('Ctrl Pts',(-21.2938985191577,19.3225217922602,-8.2387181286671));
#42474=CARTESIAN_POINT('Ctrl Pts',(-21.2868114603045,19.4313771443117,-8.2441461348259));
#42475=CARTESIAN_POINT('Ctrl Pts',(-21.2728791636074,19.5391654957492,-8.2495741409847));
#42476=CARTESIAN_POINT('Ctrl Pts',(-21.2596700733155,19.6413587017587,-8.2547203867915));
#42477=CARTESIAN_POINT('Ctrl Pts',(-21.2403084403105,19.7425933354651,-8.2598666325983));
#42478=CARTESIAN_POINT('Ctrl Pts',(-21.2149532278239,19.84224565848,-8.26501287840509));
#42479=CARTESIAN_POINT('Ctrl Pts',(-21.1943358111288,19.9232772597465,-8.26919751279814));
#42480=CARTESIAN_POINT('Ctrl Pts',(-21.1697059337058,20.0034485022604,-8.27338214719119));
#42481=CARTESIAN_POINT('Ctrl Pts',(-21.1411517779373,20.0823324956486,-8.27756678158424));
#42482=CARTESIAN_POINT('Ctrl Pts',(-21.1126382654752,20.1611042074361,-8.28174545966818));
#42483=CARTESIAN_POINT('Ctrl Pts',(-21.0802117249137,20.2385918806366,-8.28592413775212));
#42484=CARTESIAN_POINT('Ctrl Pts',(-21.04401079686,20.3143812207891,-8.29010281583607));
#42485=CARTESIAN_POINT('Ctrl Pts',(-21.0071609931882,20.391529030395,-8.2943563937215));
#42486=CARTESIAN_POINT('Ctrl Pts',(-20.9664002781982,20.466916555597,-8.29860997160694));
#42487=CARTESIAN_POINT('Ctrl Pts',(-20.9219272181894,20.5401254598066,-8.30286354949238));
#42488=CARTESIAN_POINT('Ctrl Pts',(-20.8783163552309,20.6119150665525,-8.30703466347033));
#42489=CARTESIAN_POINT('Ctrl Pts',(-20.8311360546877,20.6816093608382,-8.31120577744828));
#42490=CARTESIAN_POINT('Ctrl Pts',(-20.7806202689677,20.7488379221006,-8.31537689142623));
#42491=CARTESIAN_POINT('Ctrl Pts',(-20.7301214343074,20.8160439241699,-8.3195466057466));
#42492=CARTESIAN_POINT('Ctrl Pts',(-20.6762896134471,20.8807854689741,-8.32371632006697));
#42493=CARTESIAN_POINT('Ctrl Pts',(-20.6194012584855,20.9427222913912,-8.32788603438735));
#42494=CARTESIAN_POINT('Ctrl Pts',(-20.5625149278557,21.0046569098305,-8.33205560033139));
#42495=CARTESIAN_POINT('Ctrl Pts',(-20.5025725911954,21.0637866660879,-8.33622516627543));
#42496=CARTESIAN_POINT('Ctrl Pts',(-20.4398891227941,21.1198065121255,-8.34039473221948));
#42497=CARTESIAN_POINT('Ctrl Pts',(-20.3750017809722,21.1777959468418,-8.3447108949584));
#42498=CARTESIAN_POINT('Ctrl Pts',(-20.3071773578719,21.2324523620817,-8.34902705769732));
#42499=CARTESIAN_POINT('Ctrl Pts',(-20.2368028123897,21.2834824986169,-8.35334322043624));
#42500=CARTESIAN_POINT('Ctrl Pts',(-20.1687207103245,21.3328503338219,-8.35751878462792));
#42501=CARTESIAN_POINT('Ctrl Pts',(-20.0982524952705,21.3788242964685,-8.36169434881959));
#42502=CARTESIAN_POINT('Ctrl Pts',(-20.0257768405866,21.4211838371783,-8.36586991301127));
#42503=CARTESIAN_POINT('Ctrl Pts',(-19.949640612879,21.4656828575891,-8.37025637502381));
#42504=CARTESIAN_POINT('Ctrl Pts',(-19.8712893431908,21.5061924632349,-8.37464283703635));
#42505=CARTESIAN_POINT('Ctrl Pts',(-19.7911876038235,21.5425133219267,-8.3790292990489));
#42506=CARTESIAN_POINT('Ctrl Pts',(-19.7110858644562,21.5788341806186,-8.38341576106144));
#42507=CARTESIAN_POINT('Ctrl Pts',(-19.6292342232968,21.6109661511407,-8.38780222307398));
#42508=CARTESIAN_POINT('Ctrl Pts',(-19.5461152252309,21.638770347654,-8.39218868508653));
#42509=CARTESIAN_POINT('Ctrl Pts',(-19.4668195289777,21.6652956086964,-8.39637337892868));
#42510=CARTESIAN_POINT('Ctrl Pts',(-19.3860753481862,21.6879812201708,-8.40055807277084));
#42511=CARTESIAN_POINT('Ctrl Pts',(-19.3042893790366,21.7066702554941,-8.404742766613));
#42512=CARTESIAN_POINT('Ctrl Pts',(-19.2226201401935,21.7253326165988,-8.40892148778527));
#42513=CARTESIAN_POINT('Ctrl Pts',(-19.139912511179,21.7400096304283,-8.41310020895756));
#42514=CARTESIAN_POINT('Ctrl Pts',(-19.0565899049923,21.7505936196953,-8.41727893012983));
#42515=CARTESIAN_POINT('Ctrl Pts',(-18.9733652538744,21.7611651662959,-8.4214527387467));
#42516=CARTESIAN_POINT('Ctrl Pts',(-18.8895275166771,21.7676531957154,-8.42562654736356));
#42517=CARTESIAN_POINT('Ctrl Pts',(-18.8055104987545,21.7700010255113,-8.42980035598042));
#42518=CARTESIAN_POINT('Ctrl Pts',(-18.7215478255154,21.7723473366617,-8.43397146485485));
#42519=CARTESIAN_POINT('Ctrl Pts',(-18.6374065603104,21.7705587522904,-8.43814257372929));
#42520=CARTESIAN_POINT('Ctrl Pts',(-18.553524769967,21.7646304923274,-8.44231368260372));
#42521=CARTESIAN_POINT('Ctrl Pts',(-18.4696720738751,21.758704288571,-8.44648334473636));
#42522=CARTESIAN_POINT('Ctrl Pts',(-18.3860791323485,21.748641293549,-8.45065300686901));
#42523=CARTESIAN_POINT('Ctrl Pts',(-18.3031817775257,21.7344887872119,-8.45482266900166));
#42524=CARTESIAN_POINT('Ctrl Pts',(-18.22028830845,21.7203369442622,-8.45899213568473));
#42525=CARTESIAN_POINT('Ctrl Pts',(-18.1380908144902,21.7020960496259,-8.46316160236781));
#42526=CARTESIAN_POINT('Ctrl Pts',(-18.0570164290657,21.6798647684077,-8.46733106905089));
#42527=CARTESIAN_POINT('Ctrl Pts',(-17.9758686662976,21.6576133665023,-8.47150430935972));
#42528=CARTESIAN_POINT('Ctrl Pts',(-17.8958464874927,21.6313644844824,-8.47567754966855));
#42529=CARTESIAN_POINT('Ctrl Pts',(-17.8173628033701,21.6012669829445,-8.47985078997738));
#42530=CARTESIAN_POINT('Ctrl Pts',(-17.7388450977354,21.5711564345863,-8.48402583932395));
#42531=CARTESIAN_POINT('Ctrl Pts',(-17.6618676373455,21.5371941278435,-8.48820088867052));
#42532=CARTESIAN_POINT('Ctrl Pts',(-17.586822033013,21.4995765689746,-8.49237593801708));
#42533=CARTESIAN_POINT('Ctrl Pts',(-17.5116490489329,21.4618951593952,-8.49655807394435));
#42534=CARTESIAN_POINT('Ctrl Pts',(-17.4384148752304,21.4205463260528,-8.50074020987163));
#42535=CARTESIAN_POINT('Ctrl Pts',(-17.3674851353028,21.3757718412252,-8.50492234579891));
#42536=CARTESIAN_POINT('Ctrl Pts',(-17.3010306746449,21.3338223818942,-8.50884061178619));
#42537=CARTESIAN_POINT('Ctrl Pts',(-17.2365990013488,21.2888665194699,-8.51275887777347));
#42538=CARTESIAN_POINT('Ctrl Pts',(-17.1744642439897,21.2411350264762,-8.51667714376075));
#42539=CARTESIAN_POINT('',(-21.2939989424941,19.2086731074563,-8.16670989022852));
#42540=CARTESIAN_POINT('Ctrl Pts',(-21.2939989424941,19.2086731074563,-8.16670989022852));
#42541=CARTESIAN_POINT('Ctrl Pts',(-21.294074804776,19.2921352174732,-8.17086478789788));
#42542=CARTESIAN_POINT('Ctrl Pts',(-21.2900646933588,19.3757219830021,-8.17501968556724));
#42543=CARTESIAN_POINT('Ctrl Pts',(-21.2819596922617,19.458994771335,-8.17917458323661));
#42544=CARTESIAN_POINT('Ctrl Pts',(-21.2739328413916,19.5414646248839,-8.18328941845664));
#42545=CARTESIAN_POINT('Ctrl Pts',(-21.2618897634889,19.6236260477268,-8.18740425367667));
#42546=CARTESIAN_POINT('Ctrl Pts',(-21.2458740550218,19.7050533692914,-8.1915190888967));
#42547=CARTESIAN_POINT('Ctrl Pts',(-21.229865310909,19.7864452825742,-8.19563213480029));
#42548=CARTESIAN_POINT('Ctrl Pts',(-21.2098874553345,19.867103263636,-8.19974518070388));
#42549=CARTESIAN_POINT('Ctrl Pts',(-21.1860355605652,19.9466096857189,-8.20385822660747));
#42550=CARTESIAN_POINT('Ctrl Pts',(-21.1621864189586,20.0261069305809,-8.2079707977528));
#42551=CARTESIAN_POINT('Ctrl Pts',(-21.1344642632168,20.1044524267967,-8.21208336889812));
#42552=CARTESIAN_POINT('Ctrl Pts',(-21.1030141994638,20.1812431255818,-8.21619594004345));
#42553=CARTESIAN_POINT('Ctrl Pts',(-21.0710029255604,20.2594041147406,-8.2203818978976));
#42554=CARTESIAN_POINT('Ctrl Pts',(-21.0351295718013,20.3359537977659,-8.22456785575175));
#42555=CARTESIAN_POINT('Ctrl Pts',(-20.9955977974884,20.4104896424712,-8.22875381360589));
#42556=CARTESIAN_POINT('Ctrl Pts',(-20.9567081892514,20.4838147044139,-8.23287177349699));
#42557=CARTESIAN_POINT('Ctrl Pts',(-20.9142784405329,20.5551904907364,-8.23698973338808));
#42558=CARTESIAN_POINT('Ctrl Pts',(-20.8685472200438,20.624261534679,-8.24110769327918));
#42559=CARTESIAN_POINT('Ctrl Pts',(-20.8216832918827,20.6950433858241,-8.24532765011485));
#42560=CARTESIAN_POINT('Ctrl Pts',(-20.7713524862058,20.7634043768936,-8.24954760695052));
#42561=CARTESIAN_POINT('Ctrl Pts',(-20.7178552814756,20.8289982145112,-8.2537675637862));
#42562=CARTESIAN_POINT('Ctrl Pts',(-20.6643580767454,20.8945920521287,-8.25798752062187));
#42563=CARTESIAN_POINT('Ctrl Pts',(-20.6076948817588,20.9574183953714,-8.26220747745755));
#42564=CARTESIAN_POINT('Ctrl Pts',(-20.5482046419776,21.0171731691692,-8.26642743429322));
#42565=CARTESIAN_POINT('Ctrl Pts',(-20.4892123552949,21.0764277756309,-8.27061206868627));
#42566=CARTESIAN_POINT('Ctrl Pts',(-20.4272042190729,21.1328994502154,-8.27479670307932));
#42567=CARTESIAN_POINT('Ctrl Pts',(-20.3624734272384,21.1862656268913,-8.27898133747237));
#42568=CARTESIAN_POINT('Ctrl Pts',(-20.2978347716739,21.2395558434202,-8.28316001555632));
#42569=CARTESIAN_POINT('Ctrl Pts',(-20.2304815101078,21.2897490519969,-8.28733869364027));
#42570=CARTESIAN_POINT('Ctrl Pts',(-20.1607438576392,21.3365592122283,-8.29151737172421));
#42571=CARTESIAN_POINT('Ctrl Pts',(-20.0897562078698,21.3842084109399,-8.29577094960965));
#42572=CARTESIAN_POINT('Ctrl Pts',(-20.0162981861695,21.4283517444169,-8.30002452749509));
#42573=CARTESIAN_POINT('Ctrl Pts',(-19.9407536469185,21.4687301954948,-8.30427810538052));
#42574=CARTESIAN_POINT('Ctrl Pts',(-19.8666736859739,21.5083258315065,-8.30844921935847));
#42575=CARTESIAN_POINT('Ctrl Pts',(-19.7905878123472,21.5443010347693,-8.31262033333643));
#42576=CARTESIAN_POINT('Ctrl Pts',(-19.7128859499196,21.5764560442016,-8.31679144731438));
#42577=CARTESIAN_POINT('Ctrl Pts',(-19.6352101611023,21.60860026371,-8.32096116163475));
#42578=CARTESIAN_POINT('Ctrl Pts',(-19.5559198851418,21.6369266595076,-8.32513087595513));
#42579=CARTESIAN_POINT('Ctrl Pts',(-19.4754262787736,21.6612830598002,-8.3293005902755));
#42580=CARTESIAN_POINT('Ctrl Pts',(-19.3949355367132,21.6856385933876,-8.33347015621955));
#42581=CARTESIAN_POINT('Ctrl Pts',(-19.3132419899452,21.706024279931,-8.33763972216359));
#42582=CARTESIAN_POINT('Ctrl Pts',(-19.2307719418916,21.722337818325,-8.34180928810764));
#42583=CARTESIAN_POINT('Ctrl Pts',(-19.1454023486863,21.7392249206039,-8.34612545084656));
#42584=CARTESIAN_POINT('Ctrl Pts',(-19.0592011520722,21.7517480910506,-8.35044161358548));
#42585=CARTESIAN_POINT('Ctrl Pts',(-18.9726507026513,21.7598518674344,-8.35475777632439));
#42586=CARTESIAN_POINT('Ctrl Pts',(-18.8889196250168,21.7676916641549,-8.35893334051607));
#42587=CARTESIAN_POINT('Ctrl Pts',(-18.8048621716337,21.7713955951849,-8.36310890470776));
#42588=CARTESIAN_POINT('Ctrl Pts',(-18.7209165514638,21.770966566847,-8.36728446889944));
#42589=CARTESIAN_POINT('Ctrl Pts',(-18.632731037581,21.7705158693076,-8.37167093091198));
#42590=CARTESIAN_POINT('Ctrl Pts',(-18.5446695341427,21.7655037616187,-8.37605739292451));
#42591=CARTESIAN_POINT('Ctrl Pts',(-18.4572333890561,21.7559951361577,-8.38044385493705));
#42592=CARTESIAN_POINT('Ctrl Pts',(-18.3697972439695,21.7464865106968,-8.38483031694959));
#42593=CARTESIAN_POINT('Ctrl Pts',(-18.2829870179304,21.7324815349687,-8.38921677896213));
#42594=CARTESIAN_POINT('Ctrl Pts',(-18.1972887614195,21.7141062794818,-8.39360324097466));
#42595=CARTESIAN_POINT('Ctrl Pts',(-18.115527292268,21.6965751423758,-8.39778819867538));
#42596=CARTESIAN_POINT('Ctrl Pts',(-18.034473515681,21.6750011795361,-8.40197315637608));
#42597=CARTESIAN_POINT('Ctrl Pts',(-17.9545574583757,21.6494563404552,-8.40615811407679));
#42598=CARTESIAN_POINT('Ctrl Pts',(-17.8747749678507,21.6239541954464,-8.41033607729674));
#42599=CARTESIAN_POINT('Ctrl Pts',(-17.7961268504701,21.5944945081176,-8.41451404051668));
#42600=CARTESIAN_POINT('Ctrl Pts',(-17.719032145132,21.5612000454396,-8.41869200373662));
#42601=CARTESIAN_POINT('Ctrl Pts',(-17.6420120287322,21.5279377950727,-8.4228659247874));
#42602=CARTESIAN_POINT('Ctrl Pts',(-17.5665427606271,21.4908483161184,-8.42703984583817));
#42603=CARTESIAN_POINT('Ctrl Pts',(-17.4930266305614,21.4501036368029,-8.43121376688895));
#42604=CARTESIAN_POINT('Ctrl Pts',(-17.4195625033245,21.4093877788982,-8.43538473544887));
#42605=CARTESIAN_POINT('Ctrl Pts',(-17.3480491705109,21.3650220797705,-8.43955570400878));
#42606=CARTESIAN_POINT('Ctrl Pts',(-17.2788661013139,21.3172253765669,-8.4437266725687));
#42607=CARTESIAN_POINT('Ctrl Pts',(-17.2434387530277,21.2927495839925,-8.44586254710532));
#42608=CARTESIAN_POINT('Ctrl Pts',(-17.208622069414,21.267374832894,-8.44799842164195));
#42609=CARTESIAN_POINT('Ctrl Pts',(-17.1744642439897,21.2411350264762,-8.45013429617857));
#42610=CARTESIAN_POINT('Ctrl Pts',(-17.1732300852521,21.2427130357988,-7.65021347737832));
#42611=CARTESIAN_POINT('Ctrl Pts',(-16.6072658289841,20.7994054395201,-7.68605038744138));
#42612=CARTESIAN_POINT('Ctrl Pts',(-15.7765849789802,19.2885418340663,-7.76427923306491));
#42613=CARTESIAN_POINT('Ctrl Pts',(-16.9200888949879,16.787568930932,-7.88490001424893));
#42614=CARTESIAN_POINT('Ctrl Pts',(-19.7898863352068,16.3740305446598,-8.01207582093035));
#42615=CARTESIAN_POINT('Ctrl Pts',(-21.194097770004,17.9910561083639,-8.10601244625689));
#42616=CARTESIAN_POINT('Ctrl Pts',(-21.29615524784,19.0247813417565,-8.15755713602294));
#42617=CARTESIAN_POINT('Ctrl Pts',(-21.2944497293802,19.2086726977168,-8.16670989022852));
#42618=CARTESIAN_POINT('Origin',(-18.734,19.211,1.76670989022852));
#42619=CARTESIAN_POINT('',(-17.1744642439897,21.2411350264762,-6.8500446144235));
#42620=CARTESIAN_POINT('',(-17.1744642439897,21.2411350264762,-6.91673141505495));
#42621=CARTESIAN_POINT('',(-17.1744642439897,21.2411350264762,1.76670989022852));
#42622=CARTESIAN_POINT('',(-21.2936354886768,19.2104398261304,-7.43329008494697));
#42623=CARTESIAN_POINT('Ctrl Pts',(-17.1744642439897,21.2411350264762,-6.91673141505495));
#42624=CARTESIAN_POINT('Ctrl Pts',(-17.1077986986994,21.1899230133744,-6.92090111186911));
#42625=CARTESIAN_POINT('Ctrl Pts',(-17.0436335716999,21.1354047766269,-6.92507080868327));
#42626=CARTESIAN_POINT('Ctrl Pts',(-16.9823060367417,21.0778605355206,-6.92924050549743));
#42627=CARTESIAN_POINT('Ctrl Pts',(-16.9209802599973,21.020317944164,-6.93341008276956));
#42628=CARTESIAN_POINT('Ctrl Pts',(-16.8624922483838,20.9597498363999,-6.93757966004168));
#42629=CARTESIAN_POINT('Ctrl Pts',(-16.8071435285937,20.8964744550421,-6.94174923731381));
#42630=CARTESIAN_POINT('Ctrl Pts',(-16.7501679766327,20.8313392578402,-6.94604136850355));
#42631=CARTESIAN_POINT('Ctrl Pts',(-16.696519501211,20.7633355257695,-6.9503334996933));
#42632=CARTESIAN_POINT('Ctrl Pts',(-16.6464823621678,20.6928468583964,-6.95462563088304));
#42633=CARTESIAN_POINT('Ctrl Pts',(-16.5978036535748,20.6242718486381,-6.958801237391));
#42634=CARTESIAN_POINT('Ctrl Pts',(-16.5525428916109,20.5533455411254,-6.96297684389896));
#42635=CARTESIAN_POINT('Ctrl Pts',(-16.5109166558157,20.4804488744373,-6.96715245040692));
#42636=CARTESIAN_POINT('Ctrl Pts',(-16.4675479843273,20.4045008207689,-6.97150284393756));
#42637=CARTESIAN_POINT('Ctrl Pts',(-16.4281250493287,20.3264143312566,-6.9758532374682));
#42638=CARTESIAN_POINT('Ctrl Pts',(-16.392837789966,20.2466444883784,-6.98020363099883));
#42639=CARTESIAN_POINT('Ctrl Pts',(-16.3575505306033,20.1668746455003,-6.98455402452947));
#42640=CARTESIAN_POINT('Ctrl Pts',(-16.3263990771312,20.0854219954345,-6.98890441806011));
#42641=CARTESIAN_POINT('Ctrl Pts',(-16.2995147249235,20.0027584514457,-6.99325481159075));
#42642=CARTESIAN_POINT('Ctrl Pts',(-16.2736547230431,19.9232445622331,-6.9974394459838));
#42643=CARTESIAN_POINT('Ctrl Pts',(-16.251646255088,19.8423144298573,-7.00162408037684));
#42644=CARTESIAN_POINT('Ctrl Pts',(-16.233642830573,19.7603760326905,-7.00580871476989));
#42645=CARTESIAN_POINT('Ctrl Pts',(-16.2156650317043,19.6785542646903,-7.00998739285383));
#42646=CARTESIAN_POINT('Ctrl Pts',(-16.2016810508028,19.595727528011,-7.01416607093777));
#42647=CARTESIAN_POINT('Ctrl Pts',(-16.1917950137906,19.5123201090072,-7.01834474902171));
#42648=CARTESIAN_POINT('Ctrl Pts',(-16.1817317766699,19.4274176719615,-7.02259832690715));
#42649=CARTESIAN_POINT('Ctrl Pts',(-16.1759149888559,19.3419139888706,-7.02685190479258));
#42650=CARTESIAN_POINT('Ctrl Pts',(-16.1744002778054,19.256268776672,-7.03110548267802));
#42651=CARTESIAN_POINT('Ctrl Pts',(-16.1729149323844,19.1722839640348,-7.03527659665597));
#42652=CARTESIAN_POINT('Ctrl Pts',(-16.1755663524988,19.0881635420987,-7.03944771063393));
#42653=CARTESIAN_POINT('Ctrl Pts',(-16.1823546543812,19.00434562627,-7.04361882461188));
#42654=CARTESIAN_POINT('Ctrl Pts',(-16.1891406783834,18.9205558363523,-7.04778853893226));
#42655=CARTESIAN_POINT('Ctrl Pts',(-16.2000607901197,18.8370688090937,-7.05195825325263));
#42656=CARTESIAN_POINT('Ctrl Pts',(-16.2150630692561,18.7543198724111,-7.05612796757301));
#42657=CARTESIAN_POINT('Ctrl Pts',(-16.230064814547,18.671573880291,-7.06029753351705));
#42658=CARTESIAN_POINT('Ctrl Pts',(-16.2491483555176,18.5895663790282,-7.06446709946109));
#42659=CARTESIAN_POINT('Ctrl Pts',(-16.2722104781216,18.5087234519296,-7.06863666540513));
#42660=CARTESIAN_POINT('Ctrl Pts',(-16.2960834365062,18.4250381872446,-7.07295282814405));
#42661=CARTESIAN_POINT('Ctrl Pts',(-16.3242198111559,18.3426014204635,-7.07726899088297));
#42662=CARTESIAN_POINT('Ctrl Pts',(-16.3564491538596,18.2618677784329,-7.08158515362189));
#42663=CARTESIAN_POINT('Ctrl Pts',(-16.3876286291147,18.1837640262997,-7.08576071781358));
#42664=CARTESIAN_POINT('Ctrl Pts',(-16.4226382716204,18.1072545529911,-7.08993628200526));
#42665=CARTESIAN_POINT('Ctrl Pts',(-16.4612757941353,18.0327280941665,-7.09411184619694));
#42666=CARTESIAN_POINT('Ctrl Pts',(-16.5018648060604,17.9544374810765,-7.09849830820948));
#42667=CARTESIAN_POINT('Ctrl Pts',(-16.5464575227364,17.878335974976,-7.10288477022202));
#42668=CARTESIAN_POINT('Ctrl Pts',(-16.5947677080407,17.8048402647499,-7.10727123223456));
#42669=CARTESIAN_POINT('Ctrl Pts',(-16.643077893345,17.7313445545238,-7.11165769424711));
#42670=CARTESIAN_POINT('Ctrl Pts',(-16.6951051426578,17.6604550629257,-7.11604415625965));
#42671=CARTESIAN_POINT('Ctrl Pts',(-16.7505157350918,17.592546982189,-7.12043061827219));
#42672=CARTESIAN_POINT('Ctrl Pts',(-16.8033768040297,17.5277634529109,-7.12461525266524));
#42673=CARTESIAN_POINT('Ctrl Pts',(-16.8595134716063,17.4654518685826,-7.12879988705829));
#42674=CARTESIAN_POINT('Ctrl Pts',(-16.918665784363,17.4059621373673,-7.13298452145134));
#42675=CARTESIAN_POINT('Ctrl Pts',(-16.9777339011242,17.346557082421,-7.13716319953529));
#42676=CARTESIAN_POINT('Ctrl Pts',(-17.0398088154216,17.2899662258644,-7.14134187761924));
#42677=CARTESIAN_POINT('Ctrl Pts',(-17.1045901309627,17.2365067792763,-7.1455205557032));
#42678=CARTESIAN_POINT('Ctrl Pts',(-17.1705326050272,17.1820891105289,-7.14977413358863));
#42679=CARTESIAN_POINT('Ctrl Pts',(-17.2392791543357,17.1309165905525,-7.15402771147407));
#42680=CARTESIAN_POINT('Ctrl Pts',(-17.3104733397832,17.0832848292941,-7.1582812893595));
#42681=CARTESIAN_POINT('Ctrl Pts',(-17.3802872870217,17.0365765026735,-7.16245240333745));
#42682=CARTESIAN_POINT('Ctrl Pts',(-17.4524544129443,16.9932731384694,-7.1666235173154));
#42683=CARTESIAN_POINT('Ctrl Pts',(-17.5266063947422,16.9536119779749,-7.17079463129336));
#42684=CARTESIAN_POINT('Ctrl Pts',(-17.6007334941262,16.9139641261659,-7.17496434561372));
#42685=CARTESIAN_POINT('Ctrl Pts',(-17.6768437213085,16.8779562675928,-7.17913405993409));
#42686=CARTESIAN_POINT('Ctrl Pts',(-17.754542930911,16.8457803802159,-7.18330377425445));
#42687=CARTESIAN_POINT('Ctrl Pts',(-17.8322393756421,16.8136056377952,-7.18747334019848));
#42688=CARTESIAN_POINT('Ctrl Pts',(-17.9115242650151,16.7852627706774,-7.19164290614252));
#42689=CARTESIAN_POINT('Ctrl Pts',(-17.9919834625921,16.7608956229962,-7.19581247208655));
#42690=CARTESIAN_POINT('Ctrl Pts',(-18.075271506299,16.7356717564626,-7.20012863482547));
#42691=CARTESIAN_POINT('Ctrl Pts',(-18.1598174672101,16.7147085365435,-7.20444479756439));
#42692=CARTESIAN_POINT('Ctrl Pts',(-18.2451468157097,16.6981087241567,-7.20876096030332));
#42693=CARTESIAN_POINT('Ctrl Pts',(-18.3276965696568,16.6820496489125,-7.21293652449499));
#42694=CARTESIAN_POINT('Ctrl Pts',(-18.4109789843005,16.6700740910787,-7.21711208868666));
#42695=CARTESIAN_POINT('Ctrl Pts',(-18.4945577002227,16.6622223743376,-7.22128765287833));
#42696=CARTESIAN_POINT('Ctrl Pts',(-18.5823577783969,16.6539740860495,-7.22567411489088));
#42697=CARTESIAN_POINT('Ctrl Pts',(-18.6704842934721,16.6502772019506,-7.23006057690343));
#42698=CARTESIAN_POINT('Ctrl Pts',(-18.7584319418542,16.6511165885499,-7.23444703891598));
#42699=CARTESIAN_POINT('Ctrl Pts',(-18.8463795902362,16.6519559751493,-7.23883350092852));
#42700=CARTESIAN_POINT('Ctrl Pts',(-18.9341477974434,16.6573315210541,-7.24321996294107));
#42701=CARTESIAN_POINT('Ctrl Pts',(-19.0212404493958,16.6671657042506,-7.24760642495362));
#42702=CARTESIAN_POINT('Ctrl Pts',(-19.1043258393295,16.6765474021004,-7.25179105934667));
#42703=CARTESIAN_POINT('Ctrl Pts',(-19.1871057341706,16.6900213769478,-7.25597569373972));
#42704=CARTESIAN_POINT('Ctrl Pts',(-19.2691452086513,16.7075584477249,-7.26016032813276));
#42705=CARTESIAN_POINT('Ctrl Pts',(-19.3510679100948,16.7250705566525,-7.26433900621671));
#42706=CARTESIAN_POINT('Ctrl Pts',(-19.4322518385269,16.7466341786848,-7.26851768430066));
#42707=CARTESIAN_POINT('Ctrl Pts',(-19.5122676703941,16.7721684286898,-7.27269636238461));
#42708=CARTESIAN_POINT('Ctrl Pts',(-19.5937177285411,16.798160361775,-7.27694994027005));
#42709=CARTESIAN_POINT('Ctrl Pts',(-19.6739569228737,16.8282666158666,-7.28120351815548));
#42710=CARTESIAN_POINT('Ctrl Pts',(-19.7525437584805,16.8623474901424,-7.28545709604092));
#42711=CARTESIAN_POINT('Ctrl Pts',(-19.8296070349296,16.8957676401671,-7.28962821001887));
#42712=CARTESIAN_POINT('Ctrl Pts',(-19.9050810078235,16.9330094826423,-7.29379932399683));
#42713=CARTESIAN_POINT('Ctrl Pts',(-19.9785668286283,16.9738917305866,-7.29797043797478));
#42714=CARTESIAN_POINT('Ctrl Pts',(-20.0520279905562,17.0147602600976,-7.30214015229516));
#42715=CARTESIAN_POINT('Ctrl Pts',(-20.1235019236784,17.0592665455509,-7.30630986661553));
#42716=CARTESIAN_POINT('Ctrl Pts',(-20.1926138614937,17.1071830870871,-7.31047958093591));
#42717=CARTESIAN_POINT('Ctrl Pts',(-20.2617233400095,17.155097923547,-7.31464914687994));
#42718=CARTESIAN_POINT('Ctrl Pts',(-20.3284706127603,17.2064225119979,-7.31881871282398));
#42719=CARTESIAN_POINT('Ctrl Pts',(-20.3925105653945,17.2608864893358,-7.32298827876801));
#42720=CARTESIAN_POINT('Ctrl Pts',(-20.4588020837616,17.3172653529285,-7.32730444150693));
#42721=CARTESIAN_POINT('Ctrl Pts',(-20.5221919593123,17.3770081330231,-7.33162060424585));
#42722=CARTESIAN_POINT('Ctrl Pts',(-20.582336932496,17.4397714478444,-7.33593676698477));
#42723=CARTESIAN_POINT('Ctrl Pts',(-20.6405226895044,17.500490254287,-7.34011233117645));
#42724=CARTESIAN_POINT('Ctrl Pts',(-20.6956714299403,17.5640354429536,-7.34428789536813));
#42725=CARTESIAN_POINT('Ctrl Pts',(-20.7475130548915,17.6300619310734,-7.34846345955981));
#42726=CARTESIAN_POINT('Ctrl Pts',(-20.8019730770773,17.6994232601451,-7.35284992157235));
#42727=CARTESIAN_POINT('Ctrl Pts',(-20.8527827827185,17.771522659754,-7.35723638358489));
#42728=CARTESIAN_POINT('Ctrl Pts',(-20.8996813854342,17.8459270580721,-7.36162284559743));
#42729=CARTESIAN_POINT('Ctrl Pts',(-20.94657998815,17.9203314563902,-7.36600930760997));
#42730=CARTESIAN_POINT('Ctrl Pts',(-20.9895672706481,17.9970403100744,-7.37039576962251));
#42731=CARTESIAN_POINT('Ctrl Pts',(-21.0284398795321,18.0755945044995,-7.37478223163505));
#42732=CARTESIAN_POINT('Ctrl Pts',(-21.0682036058612,18.1559494788324,-7.37926924910127));
#42733=CARTESIAN_POINT('Ctrl Pts',(-21.103794382086,18.2385006465155,-7.38375626656748));
#42734=CARTESIAN_POINT('Ctrl Pts',(-21.1349820909848,18.3228080169409,-7.3882432840337));
#42735=CARTESIAN_POINT('Ctrl Pts',(-21.1660643193882,18.4068302499356,-7.39271512587973));
#42736=CARTESIAN_POINT('Ctrl Pts',(-21.1927730322953,18.4925965155768,-7.39718696772576));
#42737=CARTESIAN_POINT('Ctrl Pts',(-21.214925712994,18.5796462112212,-7.40165880957179));
#42738=CARTESIAN_POINT('Ctrl Pts',(-21.2370311427379,18.6665102326671,-7.40612111312312));
#42739=CARTESIAN_POINT('Ctrl Pts',(-21.2545997969947,18.7546518909174,-7.41058341667445));
#42740=CARTESIAN_POINT('Ctrl Pts',(-21.2674980351242,18.8435932689487,-7.41504572022578));
#42741=CARTESIAN_POINT('Ctrl Pts',(-21.2803582069864,18.9322721563795,-7.41949485428542));
#42742=CARTESIAN_POINT('Ctrl Pts',(-21.2885753721633,19.0217457093728,-7.42394398834505));
#42743=CARTESIAN_POINT('Ctrl Pts',(-21.292066600817,19.1115250494615,-7.42839312240469));
#42744=CARTESIAN_POINT('Ctrl Pts',(-21.2933474798424,19.1444637323838,-7.43002544244541));
#42745=CARTESIAN_POINT('Ctrl Pts',(-21.2939927168566,19.1774434535922,-7.43165776248613));
#42746=CARTESIAN_POINT('Ctrl Pts',(-21.2939999386838,19.2104396975212,-7.43329008252684));
#42747=CARTESIAN_POINT('Ctrl Pts',(-21.2898971261407,19.2104411453458,-7.4332901097715));
#42748=CARTESIAN_POINT('Ctrl Pts',(-21.2889976171803,19.6723917155128,-7.45617941928649));
#42749=CARTESIAN_POINT('Ctrl Pts',(-20.9482576239576,20.9911305382399,-7.52146066436197));
#42750=CARTESIAN_POINT('Ctrl Pts',(-19.0929372130342,22.083338204411,-7.61589315039638));
#42751=CARTESIAN_POINT('Ctrl Pts',(-17.6442977577302,21.5931891477782,-7.68743632691578));
#42752=CARTESIAN_POINT('Ctrl Pts',(-17.1756294998728,21.2395871765569,-7.7165875678747));
#42753=CARTESIAN_POINT('',(-21.2941234764334,19.2121301833364,-7.36670989022851));
#42754=CARTESIAN_POINT('Ctrl Pts',(-21.2976211331247,19.2121317273999,-7.36670989022851));
#42755=CARTESIAN_POINT('Ctrl Pts',(-21.2979709119767,19.2754624155768,-7.36987218932674));
#42756=CARTESIAN_POINT('Ctrl Pts',(-21.2671018166522,20.1874206516717,-7.41542642398545));
#42757=CARTESIAN_POINT('Ctrl Pts',(-20.178486706887,21.871216118483,-7.50337259420462));
#42758=CARTESIAN_POINT('Ctrl Pts',(-18.0960849586736,21.8671173941638,-7.594711490823));
#42759=CARTESIAN_POINT('Ctrl Pts',(-17.2767521278595,21.3237996192039,-7.6436584518809));
#42760=CARTESIAN_POINT('Ctrl Pts',(-17.1732300852521,21.2427130357988,-7.65021347737832));
#42761=CARTESIAN_POINT('Ctrl Pts',(-17.1744642439897,21.2411350264762,-6.8500446144235));
#42762=CARTESIAN_POINT('Ctrl Pts',(-17.1078662292582,21.189974889885,-6.85422898705064));
#42763=CARTESIAN_POINT('Ctrl Pts',(-17.0438781031357,21.1356032727387,-6.85841335967779));
#42764=CARTESIAN_POINT('Ctrl Pts',(-16.9828073053752,21.0783307543905,-6.86259773230493));
#42765=CARTESIAN_POINT('Ctrl Pts',(-16.9589891468458,21.0559939588775,-6.86422967513577));
#42766=CARTESIAN_POINT('Ctrl Pts',(-16.9356143137478,21.0332162880907,-6.86586161796661));
#42767=CARTESIAN_POINT('Ctrl Pts',(-16.9126993772538,21.0100175211999,-6.86749356079745));
#42768=CARTESIAN_POINT('Ctrl Pts',(-16.8539408046156,20.9505311495128,-6.8716781951905));
#42769=CARTESIAN_POINT('Ctrl Pts',(-16.7979903187279,20.8880523361676,-6.87586282958355));
#42770=CARTESIAN_POINT('Ctrl Pts',(-16.7451680193311,20.8228769657355,-6.88004746397659));
#42771=CARTESIAN_POINT('Ctrl Pts',(-16.6924209059395,20.7577943643761,-6.88422614206054));
#42772=CARTESIAN_POINT('Ctrl Pts',(-16.6427934219786,20.6900231841701,-6.88840482014448));
#42773=CARTESIAN_POINT('Ctrl Pts',(-16.5965688328439,20.6198960237255,-6.89258349822842));
#42774=CARTESIAN_POINT('Ctrl Pts',(-16.5495157011699,20.5485118843294,-6.89683707611386));
#42775=CARTESIAN_POINT('Ctrl Pts',(-16.5059889968458,20.4746868150557,-6.9010906539993));
#42776=CARTESIAN_POINT('Ctrl Pts',(-16.4662445138507,20.3988068256412,-6.90534423188473));
#42777=CARTESIAN_POINT('Ctrl Pts',(-16.4272705552135,20.324397917889,-6.90951534586268));
#42778=CARTESIAN_POINT('Ctrl Pts',(-16.3919336983952,20.2480134825273,-6.91368645984063));
#42779=CARTESIAN_POINT('Ctrl Pts',(-16.3604304325482,20.1700451024153,-6.91785757381858));
#42780=CARTESIAN_POINT('Ctrl Pts',(-16.3289377379264,20.0921028853463,-6.92202728813895));
#42781=CARTESIAN_POINT('Ctrl Pts',(-16.3012762516654,20.0125782052865,-6.92619700245933));
#42782=CARTESIAN_POINT('Ctrl Pts',(-16.2775946975111,19.9318834787289,-6.9303667167797));
#42783=CARTESIAN_POINT('Ctrl Pts',(-16.253913986048,19.8511916236359,-6.93453628272374));
#42784=CARTESIAN_POINT('Ctrl Pts',(-16.2342130538339,19.7693302464836,-6.93870584866779));
#42785=CARTESIAN_POINT('Ctrl Pts',(-16.2185906288469,19.6867264923413,-6.94287541461183));
#42786=CARTESIAN_POINT('Ctrl Pts',(-16.2024189386698,19.601218492106,-6.94719157735075));
#42787=CARTESIAN_POINT('Ctrl Pts',(-16.1906179905571,19.5149154578639,-6.95150774008967));
#42788=CARTESIAN_POINT('Ctrl Pts',(-16.1832392059578,19.4283001877063,-6.95582390282859));
#42789=CARTESIAN_POINT('Ctrl Pts',(-16.1761007844908,19.3445064008638,-6.95999946702027));
#42790=CARTESIAN_POINT('Ctrl Pts',(-16.1731008165489,19.2604208803107,-6.96417503121195));
#42791=CARTESIAN_POINT('Ctrl Pts',(-16.1742327266829,19.1764817953117,-6.96835059540363));
#42792=CARTESIAN_POINT('Ctrl Pts',(-16.1754218069069,19.0883031466757,-6.97273705741617));
#42793=CARTESIAN_POINT('Ctrl Pts',(-16.1811710990057,19.0002866979193,-6.97712351942871));
#42794=CARTESIAN_POINT('Ctrl Pts',(-16.1914115149699,18.9129332360151,-6.98150998144125));
#42795=CARTESIAN_POINT('Ctrl Pts',(-16.2016519309342,18.8255797741109,-6.9858964434538));
#42796=CARTESIAN_POINT('Ctrl Pts',(-16.2163832985703,18.7388898583324,-6.99028290546634));
#42797=CARTESIAN_POINT('Ctrl Pts',(-16.2354754819718,18.6533484665025,-6.99466936747888));
#42798=CARTESIAN_POINT('Ctrl Pts',(-16.2536892057137,18.5717429609135,-6.99885400187193));
#42799=CARTESIAN_POINT('Ctrl Pts',(-16.2759390634243,18.490878859979,-7.00303863626498));
#42800=CARTESIAN_POINT('Ctrl Pts',(-16.3021495269224,18.4111854736302,-7.00722327065803));
#42801=CARTESIAN_POINT('Ctrl Pts',(-16.3283226830699,18.3316055209528,-7.01140194874197));
#42802=CARTESIAN_POINT('Ctrl Pts',(-16.358445104793,18.2531934061978,-7.01558062682591));
#42803=CARTESIAN_POINT('Ctrl Pts',(-16.3923904554833,18.1763673400535,-7.01975930490986));
#42804=CARTESIAN_POINT('Ctrl Pts',(-16.4269442521885,18.0981642218874,-7.02401288279529));
#42805=CARTESIAN_POINT('Ctrl Pts',(-16.4654592728757,18.0216050420065,-7.02826646068073));
#42806=CARTESIAN_POINT('Ctrl Pts',(-16.5077494008732,17.9471138224161,-7.03252003856617));
#42807=CARTESIAN_POINT('Ctrl Pts',(-16.5492196522171,17.8740667604752,-7.03669115254412));
#42808=CARTESIAN_POINT('Ctrl Pts',(-16.5943197038781,17.8030086099539,-7.04086226652207));
#42809=CARTESIAN_POINT('Ctrl Pts',(-16.6428266524924,17.7343165435092,-7.04503338050002));
#42810=CARTESIAN_POINT('Ctrl Pts',(-16.6913173241316,17.6656475273508,-7.0492030948204));
#42811=CARTESIAN_POINT('Ctrl Pts',(-16.7432123571369,17.5993433939188,-7.05337280914077));
#42812=CARTESIAN_POINT('Ctrl Pts',(-16.798245475847,17.5357524295731,-7.05754252346114));
#42813=CARTESIAN_POINT('Ctrl Pts',(-16.8532766362426,17.4721637280668,-7.06171208940519));
#42814=CARTESIAN_POINT('Ctrl Pts',(-16.9114453586341,17.4112883509861,-7.06588165534924));
#42815=CARTESIAN_POINT('Ctrl Pts',(-16.9724459211976,17.3534405184612,-7.07005122129328));
#42816=CARTESIAN_POINT('Ctrl Pts',(-17.0355911882885,17.2935588275078,-7.0743673840322));
#42817=CARTESIAN_POINT('Ctrl Pts',(-17.1017707529441,17.2369219021168,-7.07868354677112));
#42818=CARTESIAN_POINT('Ctrl Pts',(-17.1706064918291,17.1838343090391,-7.08299970951004));
#42819=CARTESIAN_POINT('Ctrl Pts',(-17.2371999137602,17.132476038722,-7.08717527370172));
#42820=CARTESIAN_POINT('Ctrl Pts',(-17.3062787039752,17.0844396429708,-7.0913508378934));
#42821=CARTESIAN_POINT('Ctrl Pts',(-17.3774708722983,17.0399567655855,-7.09552640208508));
#42822=CARTESIAN_POINT('Ctrl Pts',(-17.4522587878001,16.9932271638116,-7.09991286409762));
#42823=CARTESIAN_POINT('Ctrl Pts',(-17.5293786750682,16.9504197742736,-7.10429932611016));
#42824=CARTESIAN_POINT('Ctrl Pts',(-17.6083720554812,16.9117475713793,-7.1086857881227));
#42825=CARTESIAN_POINT('Ctrl Pts',(-17.6873654358942,16.8730753684849,-7.11307225013524));
#42826=CARTESIAN_POINT('Ctrl Pts',(-17.7682317459862,16.8385385101709,-7.11745871214778));
#42827=CARTESIAN_POINT('Ctrl Pts',(-17.8504927560597,16.8082900820313,-7.12184517416032));
#42828=CARTESIAN_POINT('Ctrl Pts',(-17.9289688151197,16.7794334289094,-7.12602980855337));
#42829=CARTESIAN_POINT('Ctrl Pts',(-18.0090061529611,16.7543718340009,-7.13021444294642));
#42830=CARTESIAN_POINT('Ctrl Pts',(-18.0902029058994,16.733274167381,-7.13439907733947));
#42831=CARTESIAN_POINT('Ctrl Pts',(-18.17128408531,16.7122065306782,-7.13857775542341));
#42832=CARTESIAN_POINT('Ctrl Pts',(-18.2535209603945,16.6950917298573,-7.14275643350736));
#42833=CARTESIAN_POINT('Ctrl Pts',(-18.3364934985375,16.6820499053372,-7.1469351115913));
#42834=CARTESIAN_POINT('Ctrl Pts',(-18.4209532597953,16.6687743154856,-7.15118868947673));
#42835=CARTESIAN_POINT('Ctrl Pts',(-18.5061748645252,16.6597193207395,-7.15544226736217));
#42836=CARTESIAN_POINT('Ctrl Pts',(-18.5917010358989,16.654957941501,-7.1596958452476));
#42837=CARTESIAN_POINT('Ctrl Pts',(-18.67556911555,16.6502888708901,-7.16386695922556));
#42838=CARTESIAN_POINT('Ctrl Pts',(-18.7597295775162,16.6497484479464,-7.16803807320351));
#42839=CARTESIAN_POINT('Ctrl Pts',(-18.8437446259189,16.6533534026215,-7.17220918718146));
#42840=CARTESIAN_POINT('Ctrl Pts',(-18.9277314822607,16.6569571476192,-7.17637890150183));
#42841=CARTESIAN_POINT('Ctrl Pts',(-19.011572562719,16.6647034879404,-7.18054861582221));
#42842=CARTESIAN_POINT('Ctrl Pts',(-19.0948308836175,16.6765570486934,-7.18471833014258));
#42843=CARTESIAN_POINT('Ctrl Pts',(-19.1780862418278,16.6884101876458,-7.18888789608662));
#42844=CARTESIAN_POINT('Ctrl Pts',(-19.2607584263888,16.7043701907563,-7.19305746203067));
#42845=CARTESIAN_POINT('Ctrl Pts',(-19.3424177464726,16.7243500757491,-7.19722702797471));
#42846=CARTESIAN_POINT('Ctrl Pts',(-19.426948107513,16.7450324288504,-7.20154319071363));
#42847=CARTESIAN_POINT('Ctrl Pts',(-19.5103925419325,16.7700224760727,-7.20585935345255));
#42848=CARTESIAN_POINT('Ctrl Pts',(-19.5922902863025,16.799167131736,-7.21017551619147));
#42849=CARTESIAN_POINT('Ctrl Pts',(-19.6715202202639,16.8273624033065,-7.21435108038315));
#42850=CARTESIAN_POINT('Ctrl Pts',(-19.7493022661267,16.8594455439839,-7.21852664457483));
#42851=CARTESIAN_POINT('Ctrl Pts',(-19.8252402968867,16.8952291532946,-7.22270220876651));
#42852=CARTESIAN_POINT('Ctrl Pts',(-19.905013777055,16.9328201076442,-7.22708867077905));
#42853=CARTESIAN_POINT('Ctrl Pts',(-19.9827515495241,16.9744949002994,-7.23147513279159));
#42854=CARTESIAN_POINT('Ctrl Pts',(-20.058026370739,17.0199833023029,-7.23586159480413));
#42855=CARTESIAN_POINT('Ctrl Pts',(-20.1333011919539,17.0654717043064,-7.24024805681667));
#42856=CARTESIAN_POINT('Ctrl Pts',(-20.2061126241217,17.1147733273606,-7.24463451882921));
#42857=CARTESIAN_POINT('Ctrl Pts',(-20.2760730898188,17.1675689183003,-7.24902098084175));
#42858=CARTESIAN_POINT('Ctrl Pts',(-20.3421228419793,17.2174132934338,-7.25316224442401));
#42859=CARTESIAN_POINT('Ctrl Pts',(-20.4058887674611,17.270565700162,-7.25730350800627));
#42860=CARTESIAN_POINT('Ctrl Pts',(-20.4670153688585,17.3267872383141,-7.26144477158854));
#42861=CARTESIAN_POINT('Ctrl Pts',(-20.5280546973635,17.3829285067286,-7.26558012252323));
#42862=CARTESIAN_POINT('Ctrl Pts',(-20.5864618395734,17.4421298917808,-7.26971547345792));
#42863=CARTESIAN_POINT('Ctrl Pts',(-20.6419120481561,17.5041105435615,-7.27385082439261));
#42864=CARTESIAN_POINT('Ctrl Pts',(-20.6972986881793,17.5660201402308,-7.27798143452815));
#42865=CARTESIAN_POINT('Ctrl Pts',(-20.7497348173451,17.6307023247237,-7.28211204466368));
#42866=CARTESIAN_POINT('Ctrl Pts',(-20.7989315869956,17.6978385608179,-7.28624265479922));
#42867=CARTESIAN_POINT('Ctrl Pts',(-20.8480980593209,17.7649334517507,-7.29037072114094));
#42868=CARTESIAN_POINT('Ctrl Pts',(-20.8940288533085,17.8344790168689,-7.29449878748265));
#42869=CARTESIAN_POINT('Ctrl Pts',(-20.9364753744698,17.9061236744987,-7.29862685382437));
#42870=CARTESIAN_POINT('Ctrl Pts',(-20.9789091334294,17.9777467910562,-7.30275367899922));
#42871=CARTESIAN_POINT('Ctrl Pts',(-21.0178604599825,18.0514673424199,-7.30688050417407));
#42872=CARTESIAN_POINT('Ctrl Pts',(-21.0531249145872,18.1269060785426,-7.31100732934892));
#42873=CARTESIAN_POINT('Ctrl Pts',(-21.0883898804923,18.2023459084539,-7.31513421435873));
#42874=CARTESIAN_POINT('Ctrl Pts',(-21.1199676712092,18.2795035453347,-7.31926109936855));
#42875=CARTESIAN_POINT('Ctrl Pts',(-21.147701166054,18.3579779129534,-7.32338798437837));
#42876=CARTESIAN_POINT('Ctrl Pts',(-21.175460263615,18.4365247257135,-7.32751867920249));
#42877=CARTESIAN_POINT('Ctrl Pts',(-21.1993678247307,18.5163902510463,-7.33164937402661));
#42878=CARTESIAN_POINT('Ctrl Pts',(-21.2193162430201,18.5971570459961,-7.33578006885072));
#42879=CARTESIAN_POINT('Ctrl Pts',(-21.2392749611598,18.6779655427927,-7.33991289645234));
#42880=CARTESIAN_POINT('Ctrl Pts',(-21.2552703785523,18.7596757735081,-7.34404572405396));
#42881=CARTESIAN_POINT('Ctrl Pts',(-21.267246258349,18.8418612800574,-7.34817855165558));
#42882=CARTESIAN_POINT('Ctrl Pts',(-21.2792406903518,18.9241741027191,-7.35231778154839));
#42883=CARTESIAN_POINT('Ctrl Pts',(-21.2872031132021,19.0069632027568,-7.35645701144119));
#42884=CARTESIAN_POINT('Ctrl Pts',(-21.291129302603,19.0897988045891,-7.360596241334));
#42885=CARTESIAN_POINT('Ctrl Pts',(-21.2930622985235,19.1305815748695,-7.36263412429883));
#42886=CARTESIAN_POINT('Ctrl Pts',(-21.2940177418851,19.1713756409973,-7.36467200726367));
#42887=CARTESIAN_POINT('Ctrl Pts',(-21.2939997505486,19.2121301287168,-7.36670989022851));
#42888=CARTESIAN_POINT('Origin',(-18.734,19.211,1.76670989022852));
#42889=CARTESIAN_POINT('',(-17.1744642439897,21.2411350264762,-6.05008447538599));
#42890=CARTESIAN_POINT('',(-17.1725993531626,21.24352550386,-6.11677129344295));
#42891=CARTESIAN_POINT('',(-17.1744642439897,21.2411350264762,1.76670989022852));
#42892=CARTESIAN_POINT('',(-21.2939991231355,19.208881145288,-6.6332901097715));
#42893=CARTESIAN_POINT('Ctrl Pts',(-17.1725993531626,21.24352550386,-6.11677129344295));
#42894=CARTESIAN_POINT('Ctrl Pts',(-16.5753465248139,20.7772931197068,-6.15458085279602));
#42895=CARTESIAN_POINT('Ctrl Pts',(-15.7555914125513,19.1915608045691,-6.23478234770956));
#42896=CARTESIAN_POINT('Ctrl Pts',(-17.0342063027576,16.7062059673629,-6.35737577818358));
#42897=CARTESIAN_POINT('Ctrl Pts',(-19.9200693000182,16.4259449961135,-6.48455158486501));
#42898=CARTESIAN_POINT('Ctrl Pts',(-21.2201493011995,18.0710819511262,-6.57652302872765));
#42899=CARTESIAN_POINT('Ctrl Pts',(-21.2969229188781,19.0646440605456,-6.62610253702981));
#42900=CARTESIAN_POINT('Ctrl Pts',(-21.2956375040978,19.2088797892363,-6.6332901097715));
#42901=CARTESIAN_POINT('Ctrl Pts',(-21.2939991231355,19.208881145288,-6.6332901097715));
#42902=CARTESIAN_POINT('Ctrl Pts',(-21.2940674480299,19.2914312459012,-6.63740642252224));
#42903=CARTESIAN_POINT('Ctrl Pts',(-21.2901386830331,19.374124140816,-6.64152273527298));
#42904=CARTESIAN_POINT('Ctrl Pts',(-21.2821979940262,19.4565340775554,-6.64563904802373));
#42905=CARTESIAN_POINT('Ctrl Pts',(-21.2742662779566,19.5388508914942,-6.64975070936244));
#42906=CARTESIAN_POINT('Ctrl Pts',(-21.2623316869624,19.6208849121509,-6.65386237070115));
#42907=CARTESIAN_POINT('Ctrl Pts',(-21.2464314307688,19.7022110602224,-6.65797403203986));
#42908=CARTESIAN_POINT('Ctrl Pts',(-21.2305407999847,19.7834879765415,-6.66208320433541));
#42909=CARTESIAN_POINT('Ctrl Pts',(-21.2106893569246,19.864057405363,-6.66619237663095));
#42910=CARTESIAN_POINT('Ctrl Pts',(-21.1869659077107,19.9435013690152,-6.6703015489265));
#42911=CARTESIAN_POINT('Ctrl Pts',(-21.1632492097461,20.0229227244029,-6.67440955182855));
#42912=CARTESIAN_POINT('Ctrl Pts',(-21.1356628286736,20.1012187954781,-6.6785175547306));
#42913=CARTESIAN_POINT('Ctrl Pts',(-21.1043458531985,20.1779852823206,-6.68262555763265));
#42914=CARTESIAN_POINT('Ctrl Pts',(-21.0730277445931,20.2547545467759,-6.68673370917301));
#42915=CARTESIAN_POINT('Ctrl Pts',(-21.0379789552761,20.3299936782021,-6.69084186071338));
#42916=CARTESIAN_POINT('Ctrl Pts',(-20.9993866849092,20.4033184003596,-6.69495001225374));
#42917=CARTESIAN_POINT('Ctrl Pts',(-20.960756173379,20.4767157801412,-6.69906223457026));
#42918=CARTESIAN_POINT('Ctrl Pts',(-20.9185753946449,20.5481945435132,-6.70317445688679));
#42919=CARTESIAN_POINT('Ctrl Pts',(-20.8730771242595,20.6173957680787,-6.70728667920331));
#42920=CARTESIAN_POINT('Ctrl Pts',(-20.8275541489316,20.6866345679687,-6.71140113440066));
#42921=CARTESIAN_POINT('Ctrl Pts',(-20.7787103793541,20.7535929860942,-6.71551558959801));
#42922=CARTESIAN_POINT('Ctrl Pts',(-20.7268199445205,20.8179438909686,-6.71963004479536));
#42923=CARTESIAN_POINT('Ctrl Pts',(-20.6748438133911,20.8824010704232,-6.72375129495542));
#42924=CARTESIAN_POINT('Ctrl Pts',(-20.6198112918951,20.9442417891335,-6.72787254511548));
#42925=CARTESIAN_POINT('Ctrl Pts',(-20.5620341095488,21.003175017772,-6.73199379527554));
#42926=CARTESIAN_POINT('Ctrl Pts',(-20.5297457003867,21.0361094760174,-6.73429692959298));
#42927=CARTESIAN_POINT('Ctrl Pts',(-20.4966007367166,21.0681366118251,-6.73660006391043));
#42928=CARTESIAN_POINT('Ctrl Pts',(-20.4626578964191,21.0992112903878,-6.73890319822788));
#42929=CARTESIAN_POINT('Ctrl Pts',(-20.400986123379,21.1556718136325,-6.74308783262093));
#42930=CARTESIAN_POINT('Ctrl Pts',(-20.3364305466715,21.2092127933027,-6.74727246701397));
#42931=CARTESIAN_POINT('Ctrl Pts',(-20.2692989765722,21.2595255801518,-6.75145710140702));
#42932=CARTESIAN_POINT('Ctrl Pts',(-20.2022629599537,21.3097667529763,-6.75563577949096));
#42933=CARTESIAN_POINT('Ctrl Pts',(-20.1326585979524,21.3567885864284,-6.75981445757491));
#42934=CARTESIAN_POINT('Ctrl Pts',(-20.0608289916762,21.4003206313483,-6.76399313565885));
#42935=CARTESIAN_POINT('Ctrl Pts',(-19.9877118913305,21.4446329568875,-6.76824671354429));
#42936=CARTESIAN_POINT('Ctrl Pts',(-19.9122893426569,21.4853288288423,-6.77250029142972));
#42937=CARTESIAN_POINT('Ctrl Pts',(-19.8349567777299,21.5221672751167,-6.77675386931516));
#42938=CARTESIAN_POINT('Ctrl Pts',(-19.7591234554761,21.5582915362258,-6.78092498329311));
#42939=CARTESIAN_POINT('Ctrl Pts',(-19.6814539493099,21.5907063974351,-6.78509609727106));
#42940=CARTESIAN_POINT('Ctrl Pts',(-19.6023470115176,21.6192303601583,-6.78926721124902));
#42941=CARTESIAN_POINT('Ctrl Pts',(-19.5232666188222,21.6477447513905,-6.79343692556939));
#42942=CARTESIAN_POINT('Ctrl Pts',(-19.4427501848434,21.6723706812233,-6.79760663988977));
#42943=CARTESIAN_POINT('Ctrl Pts',(-19.3612154692014,21.6929751721551,-6.80177635421015));
#42944=CARTESIAN_POINT('Ctrl Pts',(-19.2796836549145,21.7135789298907,-6.80594592015419));
#42945=CARTESIAN_POINT('Ctrl Pts',(-19.1971340772291,21.7301614213603,-6.81011548609823));
#42946=CARTESIAN_POINT('Ctrl Pts',(-19.1139973178552,21.7426401873929,-6.81428505204228));
#42947=CARTESIAN_POINT('Ctrl Pts',(-19.027937572582,21.755557691445,-6.8186012147812));
#42948=CARTESIAN_POINT('Ctrl Pts',(-18.941249108334,21.7640774486062,-6.82291737752012));
#42949=CARTESIAN_POINT('Ctrl Pts',(-18.8544163259003,21.7681663826307,-6.82723354025904));
#42950=CARTESIAN_POINT('Ctrl Pts',(-18.7704121122212,21.7721221200595,-6.83140910445072));
#42951=CARTESIAN_POINT('Ctrl Pts',(-18.6862733092299,21.7719313177434,-6.8355846686424));
#42952=CARTESIAN_POINT('Ctrl Pts',(-18.6024375216844,21.7676171622477,-6.83976023283408));
#42953=CARTESIAN_POINT('Ctrl Pts',(-18.5143673878106,21.7630851090138,-6.84414669484662));
#42954=CARTESIAN_POINT('Ctrl Pts',(-18.4266322652435,21.7540022746856,-6.84853315685916));
#42955=CARTESIAN_POINT('Ctrl Pts',(-18.3397299608672,21.7404566879554,-6.8529196188717));
#42956=CARTESIAN_POINT('Ctrl Pts',(-18.252827656491,21.7269111012251,-6.85730608088424));
#42957=CARTESIAN_POINT('Ctrl Pts',(-18.1667587226472,21.7089029553708,-6.86169254289678));
#42958=CARTESIAN_POINT('Ctrl Pts',(-18.0820028534405,21.6865806835727,-6.86607900490932));
#42959=CARTESIAN_POINT('Ctrl Pts',(-18.0004434053584,21.6651002576761,-6.87030003908812));
#42960=CARTESIAN_POINT('Ctrl Pts',(-17.9197935149738,21.6395446599541,-6.87452107326693));
#42961=CARTESIAN_POINT('Ctrl Pts',(-17.8404904983898,21.610008288967,-6.87874210744573));
#42962=CARTESIAN_POINT('Ctrl Pts',(-17.7619934286695,21.5807720925077,-6.88292024377014));
#42963=CARTESIAN_POINT('Ctrl Pts',(-17.6848164352552,21.5476357908569,-6.88709838009456));
#42964=CARTESIAN_POINT('Ctrl Pts',(-17.6093723503702,21.5107418658815,-6.89127651641897));
#42965=CARTESIAN_POINT('Ctrl Pts',(-17.5327663637006,21.4732797437129,-6.89551899952497));
#42966=CARTESIAN_POINT('Ctrl Pts',(-17.457947583422,21.4319433870403,-6.89976148263096));
#42967=CARTESIAN_POINT('Ctrl Pts',(-17.385329256641,21.3869336446701,-6.90400396573696));
#42968=CARTESIAN_POINT('Ctrl Pts',(-17.3127109298599,21.3419239022999,-6.90824644884295));
#42969=CARTESIAN_POINT('Ctrl Pts',(-17.2422935040658,21.2932409972677,-6.91248893194895));
#42970=CARTESIAN_POINT('Ctrl Pts',(-17.1744642439897,21.2411350264762,-6.91673141505495));
#42971=CARTESIAN_POINT('',(-21.293999428374,19.2127107672549,-6.5667098902584));
#42972=CARTESIAN_POINT('Ctrl Pts',(-21.293999428374,19.2127107672549,-6.5667098902584));
#42973=CARTESIAN_POINT('Ctrl Pts',(-21.2939356382109,19.308166639887,-6.57143929947813));
#42974=CARTESIAN_POINT('Ctrl Pts',(-21.2885288437516,19.4034153336882,-6.57616870869786));
#42975=CARTESIAN_POINT('Ctrl Pts',(-21.2778724975471,19.4979019278834,-6.5808981179176));
#42976=CARTESIAN_POINT('Ctrl Pts',(-21.2671635859907,19.5928546031339,-6.58565085624617));
#42977=CARTESIAN_POINT('Ctrl Pts',(-21.2511533349013,19.6870374428281,-6.59040359457474));
#42978=CARTESIAN_POINT('Ctrl Pts',(-21.2299860493109,19.7799056526747,-6.59515633290331));
#42979=CARTESIAN_POINT('Ctrl Pts',(-21.2086961910765,19.8733116311444,-6.59993659274384));
#42980=CARTESIAN_POINT('Ctrl Pts',(-21.1821895164634,19.965387517667,-6.60471685258437));
#42981=CARTESIAN_POINT('Ctrl Pts',(-21.15066091743,20.055600503295,-6.60949711242489));
#42982=CARTESIAN_POINT('Ctrl Pts',(-21.1426476472037,20.0785289255507,-6.61071205742812));
#42983=CARTESIAN_POINT('Ctrl Pts',(-21.134310213157,20.1013371264666,-6.61192700243135));
#42984=CARTESIAN_POINT('Ctrl Pts',(-21.1256522921827,20.1240166007786,-6.61314194743458));
#42985=CARTESIAN_POINT('Ctrl Pts',(-21.0958318198279,20.2021315014283,-6.61732658182763));
#42986=CARTESIAN_POINT('Ctrl Pts',(-21.062124806143,20.2789292632222,-6.62151121622068));
#42987=CARTESIAN_POINT('Ctrl Pts',(-21.0246680532229,20.3539960060928,-6.62569585061373));
#42988=CARTESIAN_POINT('Ctrl Pts',(-20.9872646153543,20.4289559007464,-6.62987452869768));
#42989=CARTESIAN_POINT('Ctrl Pts',(-20.9461222434274,20.5021892624269,-6.63405320678162));
#42990=CARTESIAN_POINT('Ctrl Pts',(-20.9014264094923,20.5733005393213,-6.63823188486556));
#42991=CARTESIAN_POINT('Ctrl Pts',(-20.8559294348563,20.6456864347473,-6.642485462751));
#42992=CARTESIAN_POINT('Ctrl Pts',(-20.8067505255349,20.715872969927,-6.64673904063643));
#42993=CARTESIAN_POINT('Ctrl Pts',(-20.7541351457545,20.7834674854786,-6.65099261852187));
#42994=CARTESIAN_POINT('Ctrl Pts',(-20.7025398177816,20.8497515494465,-6.65516373249982));
#42995=CARTESIAN_POINT('Ctrl Pts',(-20.6476403712487,20.9135428198972,-6.65933484647777));
#42996=CARTESIAN_POINT('Ctrl Pts',(-20.5897118973506,20.9745003130228,-6.66350596045573));
#42997=CARTESIAN_POINT('Ctrl Pts',(-20.5318028619114,21.0354373512728,-6.6676756747761));
#42998=CARTESIAN_POINT('Ctrl Pts',(-20.4708671343699,21.0935421675084,-6.67184538909647));
#42999=CARTESIAN_POINT('Ctrl Pts',(-20.4072185463108,21.1485086312792,-6.67601510341685));
#43000=CARTESIAN_POINT('Ctrl Pts',(-20.3435722231416,21.2034731391074,-6.6801846693609));
#43001=CARTESIAN_POINT('Ctrl Pts',(-20.2772135801197,21.2552992164786,-6.68435423530495));
#43002=CARTESIAN_POINT('Ctrl Pts',(-20.2084905554454,21.3037201441909,-6.688523801249));
#43003=CARTESIAN_POINT('Ctrl Pts',(-20.1373513140027,21.3538434919878,-6.69283996398792));
#43004=CARTESIAN_POINT('Ctrl Pts',(-20.0636787652558,21.4003174810234,-6.69715612672683));
#43005=CARTESIAN_POINT('Ctrl Pts',(-19.9878910926204,21.4428954114938,-6.70147228946575));
#43006=CARTESIAN_POINT('Ctrl Pts',(-19.9145721954497,21.4840863703576,-6.70564785365743));
#43007=CARTESIAN_POINT('Ctrl Pts',(-19.8392743011541,21.5216310329473,-6.70982341784911));
#43008=CARTESIAN_POINT('Ctrl Pts',(-19.7623989816004,21.555353969571,-6.71399898204078));
#43009=CARTESIAN_POINT('Ctrl Pts',(-19.6816408724098,21.5907801715548,-6.71838544405332));
#43010=CARTESIAN_POINT('Ctrl Pts',(-19.5991423447412,21.6219882241026,-6.72277190606586));
#43011=CARTESIAN_POINT('Ctrl Pts',(-19.5153878511232,21.6488336748263,-6.7271583680784));
#43012=CARTESIAN_POINT('Ctrl Pts',(-19.4316333575052,21.67567912555,-6.73154483009094));
#43013=CARTESIAN_POINT('Ctrl Pts',(-19.3466234783173,21.6981618996353,-6.73593129210348));
#43014=CARTESIAN_POINT('Ctrl Pts',(-19.26085355124,21.7161996598167,-6.74031775411602));
#43015=CARTESIAN_POINT('Ctrl Pts',(-19.1790221317784,21.7334091360265,-6.7445027922189));
#43016=CARTESIAN_POINT('Ctrl Pts',(-19.0961943140709,21.746636934806,-6.74868783032178));
#43017=CARTESIAN_POINT('Ctrl Pts',(-19.0127922770448,21.7557740304907,-6.75287286842467));
#43018=CARTESIAN_POINT('Ctrl Pts',(-18.929533501023,21.764895431241,-6.75705071782109));
#43019=CARTESIAN_POINT('Ctrl Pts',(-18.8457029204263,21.7699400516436,-6.76122856721752));
#43020=CARTESIAN_POINT('Ctrl Pts',(-18.7617332667266,21.7708497740916,-6.76540641661395));
#43021=CARTESIAN_POINT('Ctrl Pts',(-18.6778456877578,21.7717586073466,-6.76958018244149));
#43022=CARTESIAN_POINT('Ctrl Pts',(-18.5938197628326,21.7685405617453,-6.77375394826903));
#43023=CARTESIAN_POINT('Ctrl Pts',(-18.5100929256421,21.7611893306287,-6.77792771409658));
#43024=CARTESIAN_POINT('Ctrl Pts',(-18.4264228070226,21.7538430794126,-6.78209865251488));
#43025=CARTESIAN_POINT('Ctrl Pts',(-18.3430518306229,21.7423692437081,-6.78626959093317));
#43026=CARTESIAN_POINT('Ctrl Pts',(-18.2604156415009,21.7268135573577,-6.79044052935147));
#43027=CARTESIAN_POINT('Ctrl Pts',(-18.1778106423785,21.7112637423073,-6.79460989350105));
#43028=CARTESIAN_POINT('Ctrl Pts',(-18.095940330876,21.6916352235908,-6.79877925765063));
#43029=CARTESIAN_POINT('Ctrl Pts',(-18.0152320947977,21.668025172531,-6.8029486218002));
#43030=CARTESIAN_POINT('Ctrl Pts',(-17.9344957178936,21.6444068892713,-6.80711943969671));
#43031=CARTESIAN_POINT('Ctrl Pts',(-17.8549226701451,21.6168044215289,-6.81129025759322));
#43032=CARTESIAN_POINT('Ctrl Pts',(-17.7769262677244,21.5853651511484,-6.81546107548973));
#43033=CARTESIAN_POINT('Ctrl Pts',(-17.6989179895601,21.5539210938201,-6.81963252843557));
#43034=CARTESIAN_POINT('Ctrl Pts',(-17.6224872571105,21.5186392540143,-6.82380398138141));
#43035=CARTESIAN_POINT('Ctrl Pts',(-17.5480265683683,21.4797148387278,-6.82797543432725));
#43036=CARTESIAN_POINT('Ctrl Pts',(-17.4734822892922,21.4407467264929,-6.83215157018901));
#43037=CARTESIAN_POINT('Ctrl Pts',(-17.4009128736038,21.3981280959147,-6.83632770605077));
#43038=CARTESIAN_POINT('Ctrl Pts',(-17.3306849632431,21.3520994623352,-6.84050384191253));
#43039=CARTESIAN_POINT('Ctrl Pts',(-17.2772042226053,21.3170472245321,-6.84368409941619));
#43040=CARTESIAN_POINT('Ctrl Pts',(-17.2250808728016,21.2800183723873,-6.84686435691984));
#43041=CARTESIAN_POINT('Ctrl Pts',(-17.1744642439897,21.2411350264762,-6.8500446144235));
#43042=CARTESIAN_POINT('Ctrl Pts',(-17.1744642439897,21.2411350264762,-6.05008447538598));
#43043=CARTESIAN_POINT('Ctrl Pts',(-17.1077758011212,21.1899054236124,-6.05425481627113));
#43044=CARTESIAN_POINT('Ctrl Pts',(-17.0436322849344,21.1354002166438,-6.05842515715628));
#43045=CARTESIAN_POINT('Ctrl Pts',(-16.9823603368735,21.0779114843939,-6.06259549804143));
#43046=CARTESIAN_POINT('Ctrl Pts',(-16.9210197564991,21.0203583575097,-6.06677051023461));
#43047=CARTESIAN_POINT('Ctrl Pts',(-16.8625574985143,20.9598153519561,-6.07094552242779));
#43048=CARTESIAN_POINT('Ctrl Pts',(-16.8072633791422,20.8966114599294,-6.07512053462096));
#43049=CARTESIAN_POINT('Ctrl Pts',(-16.7519330537637,20.8333661826606,-6.0792982805681));
#43050=CARTESIAN_POINT('Ctrl Pts',(-16.6997752805568,20.767456911828,-6.08347602651524));
#43051=CARTESIAN_POINT('Ctrl Pts',(-16.6510381296659,20.6992438801266,-6.08765377246238));
#43052=CARTESIAN_POINT('Ctrl Pts',(-16.6022223963696,20.6309208636598,-6.09183825448907));
#43053=CARTESIAN_POINT('Ctrl Pts',(-16.5568385388414,20.5602870604179,-6.09602273651575));
#43054=CARTESIAN_POINT('Ctrl Pts',(-16.5150897902318,20.4877292120832,-6.10020721854244));
#43055=CARTESIAN_POINT('Ctrl Pts',(-16.5010171667419,20.4632714902385,-6.10161771926458));
#43056=CARTESIAN_POINT('Ctrl Pts',(-16.4873571727183,20.4385953340331,-6.10302821998671));
#43057=CARTESIAN_POINT('Ctrl Pts',(-16.4741163568267,20.4137160593082,-6.10443872070885));
#43058=CARTESIAN_POINT('Ctrl Pts',(-16.4348338717473,20.3399049175952,-6.1086233551019));
#43059=CARTESIAN_POINT('Ctrl Pts',(-16.3990982578627,20.2640298565514,-6.11280798949495));
#43060=CARTESIAN_POINT('Ctrl Pts',(-16.3671315774457,20.1864659759906,-6.116992623888));
#43061=CARTESIAN_POINT('Ctrl Pts',(-16.3352103976415,20.1090124980131,-6.12117130197196));
#43062=CARTESIAN_POINT('Ctrl Pts',(-16.3070476692931,20.0298753969617,-6.12534998005591));
#43063=CARTESIAN_POINT('Ctrl Pts',(-16.2828196558214,19.949454413158,-6.12952865813987));
#43064=CARTESIAN_POINT('Ctrl Pts',(-16.2581573726207,19.8675919410174,-6.1337822360253));
#43065=CARTESIAN_POINT('Ctrl Pts',(-16.2375724777941,19.7843995318231,-6.13803581391074));
#43066=CARTESIAN_POINT('Ctrl Pts',(-16.2211996301976,19.7003202443399,-6.14228939179617));
#43067=CARTESIAN_POINT('Ctrl Pts',(-16.2051442022007,19.6178709979118,-6.14646050577412));
#43068=CARTESIAN_POINT('Ctrl Pts',(-16.1931390533221,19.5345694264037,-6.15063161975207));
#43069=CARTESIAN_POINT('Ctrl Pts',(-16.18526042222,19.4508469609104,-6.15480273373002));
#43070=CARTESIAN_POINT('Ctrl Pts',(-16.1773844348688,19.367152589299,-6.1589724480504));
#43071=CARTESIAN_POINT('Ctrl Pts',(-16.1736322583368,19.2830380618256,-6.16314216237078));
#43072=CARTESIAN_POINT('Ctrl Pts',(-16.1740284019004,19.1989411060445,-6.16731187669115));
#43073=CARTESIAN_POINT('Ctrl Pts',(-16.1744245313676,19.114847142794,-6.17148144263519));
#43074=CARTESIAN_POINT('Ctrl Pts',(-16.1789686844147,19.0307712100162,-6.17565100857924));
#43075=CARTESIAN_POINT('Ctrl Pts',(-16.187633250542,18.9471508437487,-6.17982057452328));
#43076=CARTESIAN_POINT('Ctrl Pts',(-16.1966024521254,18.8605904885601,-6.1841367372622));
#43077=CARTESIAN_POINT('Ctrl Pts',(-16.2099871509034,18.7745188559838,-6.18845290000111));
#43078=CARTESIAN_POINT('Ctrl Pts',(-16.2276984844483,18.6894132736129,-6.19276906274003));
#43079=CARTESIAN_POINT('Ctrl Pts',(-16.2448328731659,18.6070799966362,-6.19694462693171));
#43080=CARTESIAN_POINT('Ctrl Pts',(-16.2660161808879,18.5256512422045,-6.20112019112339));
#43081=CARTESIAN_POINT('Ctrl Pts',(-16.291116741615,18.4455449811371,-6.20529575531507));
#43082=CARTESIAN_POINT('Ctrl Pts',(-16.3174850719936,18.3613927432578,-6.20968221732761));
#43083=CARTESIAN_POINT('Ctrl Pts',(-16.3481765728437,18.2787006554449,-6.21406867934014));
#43084=CARTESIAN_POINT('Ctrl Pts',(-16.3829817631983,18.1979288029829,-6.21845514135268));
#43085=CARTESIAN_POINT('Ctrl Pts',(-16.4177869535528,18.117156950521,-6.22284160336521));
#43086=CARTESIAN_POINT('Ctrl Pts',(-16.4567055084016,18.0383058200372,-6.22722806537775));
#43087=CARTESIAN_POINT('Ctrl Pts',(-16.4994739740983,17.9618028820207,-6.23161452739028));
#43088=CARTESIAN_POINT('Ctrl Pts',(-16.5402745992903,17.8888199575868,-6.23579916178333));
#43089=CARTESIAN_POINT('Ctrl Pts',(-16.5847305081231,17.8177022301347,-6.23998379617638));
#43090=CARTESIAN_POINT('Ctrl Pts',(-16.6326464991108,17.7488394533087,-6.24416843056943));
#43091=CARTESIAN_POINT('Ctrl Pts',(-16.6804942876163,17.6800746941218,-6.24834710865338));
#43092=CARTESIAN_POINT('Ctrl Pts',(-16.7317921151762,17.6135588845839,-6.25252578673734));
#43093=CARTESIAN_POINT('Ctrl Pts',(-16.7862992714868,17.5496566061921,-6.2567044648213));
#43094=CARTESIAN_POINT('Ctrl Pts',(-16.8417834294006,17.4846089253861,-6.26095804270673));
#43095=CARTESIAN_POINT('Ctrl Pts',(-16.9005928669026,17.4222698132391,-6.26521162059216));
#43096=CARTESIAN_POINT('Ctrl Pts',(-16.9624279299719,17.3629923158449,-6.2694651984776));
#43097=CARTESIAN_POINT('Ctrl Pts',(-17.0230641996824,17.3048640284082,-6.27363631245555));
#43098=CARTESIAN_POINT('Ctrl Pts',(-17.0866094791688,17.2496800373392,-6.2778074264335));
#43099=CARTESIAN_POINT('Ctrl Pts',(-17.1527422696958,17.1977379727534,-6.28197854041145));
#43100=CARTESIAN_POINT('Ctrl Pts',(-17.2188528687262,17.145813337829,-6.28614825473182));
#43101=CARTESIAN_POINT('Ctrl Pts',(-17.2875488929276,17.0971287527973,-6.2903179690522));
#43102=CARTESIAN_POINT('Ctrl Pts',(-17.3584755491053,17.0519417597039,-6.29448768337257));
#43103=CARTESIAN_POINT('Ctrl Pts',(-17.429399681408,17.0067563745576,-6.29865724931661));
#43104=CARTESIAN_POINT('Ctrl Pts',(-17.5025538994269,16.965068580356,-6.30282681526065));
#43105=CARTESIAN_POINT('Ctrl Pts',(-17.5775553595561,16.9270919909969,-6.30699638120468));
#43106=CARTESIAN_POINT('Ctrl Pts',(-17.6551937784993,16.887780191605,-6.3113125439436));
#43107=CARTESIAN_POINT('Ctrl Pts',(-17.7348112839525,16.8524456628668,-6.31562870668252));
#43108=CARTESIAN_POINT('Ctrl Pts',(-17.8159584194019,16.8212720539164,-6.31994486942144));
#43109=CARTESIAN_POINT('Ctrl Pts',(-17.8944621954492,16.7911139219987,-6.32412043361312));
#43110=CARTESIAN_POINT('Ctrl Pts',(-17.9743970142431,16.7648498911064,-6.3282959978048));
#43111=CARTESIAN_POINT('Ctrl Pts',(-18.055340160162,16.7425954906477,-6.33247156199648));
#43112=CARTESIAN_POINT('Ctrl Pts',(-18.1403715519571,16.7192170733266,-6.33685802400902));
#43113=CARTESIAN_POINT('Ctrl Pts',(-18.2265152388011,16.7002641097526,-6.34124448602156));
#43114=CARTESIAN_POINT('Ctrl Pts',(-18.3132709737052,16.6858094950216,-6.3456309480341));
#43115=CARTESIAN_POINT('Ctrl Pts',(-18.4000267086093,16.6713548802907,-6.35001741004664));
#43116=CARTESIAN_POINT('Ctrl Pts',(-18.4873939064752,16.6613986045227,-6.35440387205918));
#43117=CARTESIAN_POINT('Ctrl Pts',(-18.5748705298082,16.6559505265619,-6.35879033407172));
#43118=CARTESIAN_POINT('Ctrl Pts',(-18.6583222240303,16.650753122744,-6.36297496846477));
#43119=CARTESIAN_POINT('Ctrl Pts',(-18.7421841184714,16.6496388297569,-6.36715960285782));
#43120=CARTESIAN_POINT('Ctrl Pts',(-18.8260228331344,16.6526544802975,-6.37134423725087));
#43121=CARTESIAN_POINT('Ctrl Pts',(-18.909742213764,16.6556658384328,-6.3755229153348));
#43122=CARTESIAN_POINT('Ctrl Pts',(-18.9934380243477,16.6627954472227,-6.37970159341873));
#43123=CARTESIAN_POINT('Ctrl Pts',(-19.0766734176208,16.6740382484444,-6.38388027150266));
#43124=CARTESIAN_POINT('Ctrl Pts',(-19.1614007454985,16.685482568798,-6.38813384938809));
#43125=CARTESIAN_POINT('Ctrl Pts',(-19.2456505065464,16.7011890198916,-6.39238742727353));
#43126=CARTESIAN_POINT('Ctrl Pts',(-19.3289636478323,16.7210967372691,-6.39664100515897));
#43127=CARTESIAN_POINT('Ctrl Pts',(-19.4106616013021,16.7406185046985,-6.40081211913691));
#43128=CARTESIAN_POINT('Ctrl Pts',(-19.4914584592896,16.7641799807696,-6.40498323311487));
#43129=CARTESIAN_POINT('Ctrl Pts',(-19.570929940801,16.7916719374606,-6.40915434709281));
#43130=CARTESIAN_POINT('Ctrl Pts',(-19.6503747548893,16.81915466896,-6.41332406141319));
#43131=CARTESIAN_POINT('Ctrl Pts',(-19.7284946413755,16.8505651114304,-6.41749377573357));
#43132=CARTESIAN_POINT('Ctrl Pts',(-19.804881005329,16.8857443425667,-6.42166349005394));
#43133=CARTESIAN_POINT('Ctrl Pts',(-19.8812646511277,16.920922321875,-6.42583305599798));
#43134=CARTESIAN_POINT('Ctrl Pts',(-19.9559144795488,16.959868629993,-6.43000262194201));
#43135=CARTESIAN_POINT('Ctrl Pts',(-20.028443649127,17.0023769811861,-6.43417218788604));
#43136=CARTESIAN_POINT('Ctrl Pts',(-20.1035228548334,17.0463798735676,-6.43848835062497));
#43137=CARTESIAN_POINT('Ctrl Pts',(-20.1763290473284,17.0941996856767,-6.44280451336389));
#43138=CARTESIAN_POINT('Ctrl Pts',(-20.2464645244668,17.1455579015065,-6.44712067610282));
#43139=CARTESIAN_POINT('Ctrl Pts',(-20.3143153458142,17.1952431288574,-6.45129624029449));
#43140=CARTESIAN_POINT('Ctrl Pts',(-20.379666440751,17.2482394397184,-6.45547180448617));
#43141=CARTESIAN_POINT('Ctrl Pts',(-20.4421918593792,17.3042539310253,-6.45964736867784));
#43142=CARTESIAN_POINT('Ctrl Pts',(-20.5078752882625,17.3630975811265,-6.46403383069039));
#43143=CARTESIAN_POINT('Ctrl Pts',(-20.5704396751013,17.4252719095171,-6.46842029270294));
#43144=CARTESIAN_POINT('Ctrl Pts',(-20.6295529524488,17.4903957443785,-6.47280675471549));
#43145=CARTESIAN_POINT('Ctrl Pts',(-20.6886662297962,17.5555195792399,-6.47719321672804));
#43146=CARTESIAN_POINT('Ctrl Pts',(-20.7443280892572,17.623592423249,-6.48157967874059));
#43147=CARTESIAN_POINT('Ctrl Pts',(-20.7962584977302,17.6941974787272,-6.48596614075314));
#43148=CARTESIAN_POINT('Ctrl Pts',(-20.8460908704134,17.7619500256716,-6.4901753857061));
#43149=CARTESIAN_POINT('Ctrl Pts',(-20.8926734978045,17.8322867639503,-6.49438463065905));
#43150=CARTESIAN_POINT('Ctrl Pts',(-20.9357293738867,17.9048653345981,-6.498593875612));
#43151=CARTESIAN_POINT('Ctrl Pts',(-20.9787228581407,17.9773387323842,-6.5027970209913));
#43152=CARTESIAN_POINT('Ctrl Pts',(-21.0181995127222,18.0520471246587,-6.50700016637059));
#43153=CARTESIAN_POINT('Ctrl Pts',(-21.0539239335172,18.1286170073888,-6.51120331174989));
#43154=CARTESIAN_POINT('Ctrl Pts',(-21.0896068791136,18.2050979943154,-6.51540157737787));
#43155=CARTESIAN_POINT('Ctrl Pts',(-21.1215460556625,18.283435770082,-6.51959984300585));
#43156=CARTESIAN_POINT('Ctrl Pts',(-21.1495512259746,18.3632310015738,-6.52379810863383));
#43157=CARTESIAN_POINT('Ctrl Pts',(-21.177530608527,18.4429527559101,-6.52799250840905));
#43158=CARTESIAN_POINT('Ctrl Pts',(-21.20158303815,18.5241288717761,-6.53218690818426));
#43159=CARTESIAN_POINT('Ctrl Pts',(-21.2215663308331,18.6063399717978,-6.53638130795947));
#43160=CARTESIAN_POINT('Ctrl Pts',(-21.2415389226779,18.6885070486596,-6.54057346167871));
#43161=CARTESIAN_POINT('Ctrl Pts',(-21.2574466025638,18.7717075687081,-6.54476561539795));
#43162=CARTESIAN_POINT('Ctrl Pts',(-21.2691973211302,18.8555080269057,-6.54895776911719));
#43163=CARTESIAN_POINT('Ctrl Pts',(-21.2809466969547,18.9392989093157,-6.55314944380356));
#43164=CARTESIAN_POINT('Ctrl Pts',(-21.288539988214,19.0236891460417,-6.55734111848993));
#43165=CARTESIAN_POINT('Ctrl Pts',(-21.2919366299884,19.1082371810269,-6.5615327931763));
#43166=CARTESIAN_POINT('Ctrl Pts',(-21.2933350165072,19.1430453357178,-6.56325849219371));
#43167=CARTESIAN_POINT('Ctrl Pts',(-21.294022704555,19.1778801783151,-6.56498419121111));
#43168=CARTESIAN_POINT('Ctrl Pts',(-21.2939994283744,19.2127107666517,-6.56670989022851));
#43169=CARTESIAN_POINT('Origin',(-18.734,19.211,1.76670989022852));
#43170=CARTESIAN_POINT('',(-17.1744642439897,21.2411350264762,-5.25018233500805));
#43171=CARTESIAN_POINT('',(-17.1744642439897,21.2411350264762,-5.31661774316889));
#43172=CARTESIAN_POINT('',(-17.1744642439897,21.2411350264762,1.76670989022852));
#43173=CARTESIAN_POINT('',(-21.2939994369002,19.2126979607666,-5.8332901097715));
#43174=CARTESIAN_POINT('Ctrl Pts',(-17.1744642439897,21.2411350264762,-5.31661774316889));
#43175=CARTESIAN_POINT('Ctrl Pts',(-17.1078004643465,21.1899243697324,-5.32080131395071));
#43176=CARTESIAN_POINT('Ctrl Pts',(-17.043740061828,21.1354869082706,-5.32498488473253));
#43177=CARTESIAN_POINT('Ctrl Pts',(-16.9825942508179,21.0781309278494,-5.32916845551436));
#43178=CARTESIAN_POINT('Ctrl Pts',(-16.9299734999191,21.0287716224703,-5.33276874525361));
#43179=CARTESIAN_POINT('Ctrl Pts',(-16.8795107939483,20.9772516236668,-5.33636903499286));
#43180=CARTESIAN_POINT('Ctrl Pts',(-16.8313804354228,20.923786849695,-5.3399693247321));
#43181=CARTESIAN_POINT('Ctrl Pts',(-16.7754382840342,20.8616444811128,-5.34415395912515));
#43182=CARTESIAN_POINT('Ctrl Pts',(-16.7224397206528,20.7966428559978,-5.3483385935182));
#43183=CARTESIAN_POINT('Ctrl Pts',(-16.6726908063355,20.7290923582293,-5.35252322791125));
#43184=CARTESIAN_POINT('Ctrl Pts',(-16.6230127034401,20.6616380102332,-5.35670190599519));
#43185=CARTESIAN_POINT('Ctrl Pts',(-16.5765753324319,20.5916423631924,-5.36088058407914));
#43186=CARTESIAN_POINT('Ctrl Pts',(-16.533646260122,20.5194507707227,-5.36505926216308));
#43187=CARTESIAN_POINT('Ctrl Pts',(-16.4899477150435,20.4459651958412,-5.36931284004852));
#43188=CARTESIAN_POINT('Ctrl Pts',(-16.4498848008428,20.3702045348863,-5.37356641793395));
#43189=CARTESIAN_POINT('Ctrl Pts',(-16.4136951701205,20.2925662237874,-5.37781999581939));
#43190=CARTESIAN_POINT('Ctrl Pts',(-16.378207146008,20.2164330828479,-5.38199110979734));
#43191=CARTESIAN_POINT('Ctrl Pts',(-16.3464437665668,20.1384948820616,-5.38616222377529));
#43192=CARTESIAN_POINT('Ctrl Pts',(-16.3185831851716,20.0591518794675,-5.39033333775325));
#43193=CARTESIAN_POINT('Ctrl Pts',(-16.2907319526636,19.9798355011843,-5.39450305207362));
#43194=CARTESIAN_POINT('Ctrl Pts',(-16.2667810695588,19.8991156909809,-5.39867276639399));
#43195=CARTESIAN_POINT('Ctrl Pts',(-16.2468600106956,19.8174113072849,-5.40284248071437));
#43196=CARTESIAN_POINT('Ctrl Pts',(-16.2269396607092,19.7357098309815,-5.40701204665841));
#43197=CARTESIAN_POINT('Ctrl Pts',(-16.2110489579958,19.6530242979866,-5.41118161260245));
#43198=CARTESIAN_POINT('Ctrl Pts',(-16.1992667534716,19.5697859653661,-5.4153511785465));
#43199=CARTESIAN_POINT('Ctrl Pts',(-16.1870703011714,19.4836210756563,-5.41966734128542));
#43200=CARTESIAN_POINT('Ctrl Pts',(-16.1792767060087,19.3968643124029,-5.42398350402434));
#43201=CARTESIAN_POINT('Ctrl Pts',(-16.1759149870658,19.3100003363692,-5.42829966676326));
#43202=CARTESIAN_POINT('Ctrl Pts',(-16.1726627757638,19.2259659452184,-5.43247523095494));
#43203=CARTESIAN_POINT('Ctrl Pts',(-16.1735580857934,19.1418316894465,-5.43665079514662));
#43204=CARTESIAN_POINT('Ctrl Pts',(-16.1785740672325,19.0580349643242,-5.4408263593383));
#43205=CARTESIAN_POINT('Ctrl Pts',(-16.1838433939698,18.9700058658238,-5.44521282135084));
#43206=CARTESIAN_POINT('Ctrl Pts',(-16.1936605371381,18.8823498716687,-5.44959928336338));
#43207=CARTESIAN_POINT('Ctrl Pts',(-16.2079333028748,18.7955640342066,-5.45398574537592));
#43208=CARTESIAN_POINT('Ctrl Pts',(-16.2222060686114,18.7087781967444,-5.45837220738847));
#43209=CARTESIAN_POINT('Ctrl Pts',(-16.2409342590202,18.6228630666792,-5.46275866940101));
#43210=CARTESIAN_POINT('Ctrl Pts',(-16.2639654295305,18.5382970784325,-5.46714513141355));
#43211=CARTESIAN_POINT('Ctrl Pts',(-16.2859369017452,18.4576220966618,-5.47132976580659));
#43212=CARTESIAN_POINT('Ctrl Pts',(-16.3119058645756,18.377874545241,-5.47551440019964));
#43213=CARTESIAN_POINT('Ctrl Pts',(-16.3417769993438,18.299479777991,-5.47969903459269));
#43214=CARTESIAN_POINT('Ctrl Pts',(-16.3716056162489,18.2211965959888,-5.48387771267663));
#43215=CARTESIAN_POINT('Ctrl Pts',(-16.4053252101866,18.1442627996736,-5.48805639076058));
#43216=CARTESIAN_POINT('Ctrl Pts',(-16.4427902222593,18.0690903037519,-5.49223506884452));
#43217=CARTESIAN_POINT('Ctrl Pts',(-16.4809267677478,17.9925703948664,-5.49648864672995));
#43218=CARTESIAN_POINT('Ctrl Pts',(-16.5229441986227,17.9178760152569,-5.50074222461539));
#43219=CARTESIAN_POINT('Ctrl Pts',(-16.5686369710084,17.8454221176819,-5.50499580250083));
#43220=CARTESIAN_POINT('Ctrl Pts',(-16.6134438998393,17.7743728802935,-5.50916691647878));
#43221=CARTESIAN_POINT('Ctrl Pts',(-16.6617846778615,17.7054784349765,-5.51333803045673));
#43222=CARTESIAN_POINT('Ctrl Pts',(-16.7134191824492,17.6391052326107,-5.51750914443468));
#43223=CARTESIAN_POINT('Ctrl Pts',(-16.7650363605803,17.572754302414,-5.52167885875505));
#43224=CARTESIAN_POINT('Ctrl Pts',(-16.8199447880143,17.5089232977414,-5.52584857307543));
#43225=CARTESIAN_POINT('Ctrl Pts',(-16.8778623533736,17.4479478065649,-5.5300182873958));
#43226=CARTESIAN_POINT('Ctrl Pts',(-16.9357778577775,17.386974485158,-5.53418785333984));
#43227=CARTESIAN_POINT('Ctrl Pts',(-16.9967019697692,17.3288568081793,-5.53835741928389));
#43228=CARTESIAN_POINT('Ctrl Pts',(-17.0603147509096,17.2738945080412,-5.54252698522793));
#43229=CARTESIAN_POINT('Ctrl Pts',(-17.12616407896,17.2169998012335,-5.54684314796685));
#43230=CARTESIAN_POINT('Ctrl Pts',(-17.1948942620563,17.1634868305881,-5.55115931070577));
#43231=CARTESIAN_POINT('Ctrl Pts',(-17.2661134846746,17.1136423342391,-5.55547547344469));
#43232=CARTESIAN_POINT('Ctrl Pts',(-17.3350127486071,17.0654215171161,-5.55965103763637));
#43233=CARTESIAN_POINT('Ctrl Pts',(-17.4062409575146,17.0206340542482,-5.56382660182805));
#43234=CARTESIAN_POINT('Ctrl Pts',(-17.4794157978406,16.9794941228641,-5.56800216601973));
#43235=CARTESIAN_POINT('Ctrl Pts',(-17.5562865253948,16.9362763113467,-5.57238862803227));
#43236=CARTESIAN_POINT('Ctrl Pts',(-17.6353051780176,16.897084448046,-5.57677509004481));
#43237=CARTESIAN_POINT('Ctrl Pts',(-17.7160039105555,16.8621100575217,-5.58116155205735));
#43238=CARTESIAN_POINT('Ctrl Pts',(-17.7967026430934,16.8271356669974,-5.58554801406989));
#43239=CARTESIAN_POINT('Ctrl Pts',(-17.8790808853742,16.7963788809358,-5.58993447608243));
#43240=CARTESIAN_POINT('Ctrl Pts',(-17.9626538344085,16.7699704850561,-5.59432093809497));
#43241=CARTESIAN_POINT('Ctrl Pts',(-18.0423814681728,16.7447771786174,-5.59850557248802));
#43242=CARTESIAN_POINT('Ctrl Pts',(-18.1234930456338,16.7234471296282,-5.60269020688106));
#43243=CARTESIAN_POINT('Ctrl Pts',(-18.2055793173493,16.7061304261206,-5.60687484127411));
#43244=CARTESIAN_POINT('Ctrl Pts',(-18.2875487494172,16.688838370797,-5.61105351935805));
#43245=CARTESIAN_POINT('Ctrl Pts',(-18.370489673737,16.6755484082766,-5.61523219744199));
#43246=CARTESIAN_POINT('Ctrl Pts',(-18.4539769469565,16.6663611081798,-5.61941087552594));
#43247=CARTESIAN_POINT('Ctrl Pts',(-18.5389606695472,16.6570091323315,-5.62366445341137));
#43248=CARTESIAN_POINT('Ctrl Pts',(-18.624510060566,16.6519084913031,-5.62791803129681));
#43249=CARTESIAN_POINT('Ctrl Pts',(-18.7101649534091,16.6511109612809,-5.63217160918225));
#43250=CARTESIAN_POINT('Ctrl Pts',(-18.7941592590127,16.6503288929346,-5.6363427231602));
#43251=CARTESIAN_POINT('Ctrl Pts',(-18.87825453103,16.6536845805936,-5.64051383713815));
#43252=CARTESIAN_POINT('Ctrl Pts',(-18.9620126684402,16.6611744720411,-5.6446849511161));
#43253=CARTESIAN_POINT('Ctrl Pts',(-19.0457426999984,16.6686618501832,-5.64885466543648));
#43254=CARTESIAN_POINT('Ctrl Pts',(-19.1291353638019,16.6802806360297,-5.65302437975685));
#43255=CARTESIAN_POINT('Ctrl Pts',(-19.2117557819362,16.6959752659613,-5.65719409407723));
#43256=CARTESIAN_POINT('Ctrl Pts',(-19.2943732600815,16.7116693374106,-5.66136366002127));
#43257=CARTESIAN_POINT('Ctrl Pts',(-19.3762180954027,16.7314388778862,-5.66553322596532));
#43258=CARTESIAN_POINT('Ctrl Pts',(-19.4568650837658,16.7551771092621,-5.66970279190936));
#43259=CARTESIAN_POINT('Ctrl Pts',(-19.5403475207509,16.7797499475689,-5.67401895464828));
#43260=CARTESIAN_POINT('Ctrl Pts',(-19.6225458049915,16.808575598709,-5.6783351173872));
#43261=CARTESIAN_POINT('Ctrl Pts',(-19.7030067527823,16.8414798137466,-5.68265128012612));
#43262=CARTESIAN_POINT('Ctrl Pts',(-19.7808466936618,16.8733121774403,-5.6868268443178));
#43263=CARTESIAN_POINT('Ctrl Pts',(-19.8570603406959,16.9089612248342,-5.69100240850948));
#43264=CARTESIAN_POINT('Ctrl Pts',(-19.9312606656524,16.9482214208011,-5.69517797270116));
#43265=CARTESIAN_POINT('Ctrl Pts',(-20.009208672628,16.989464555934,-5.6995644347137));
#43266=CARTESIAN_POINT('Ctrl Pts',(-20.0849341253746,17.0346929255447,-5.70395089672624));
#43267=CARTESIAN_POINT('Ctrl Pts',(-20.1580227463385,17.0836168145088,-5.70833735873878));
#43268=CARTESIAN_POINT('Ctrl Pts',(-20.2311113673024,17.1325407034729,-5.71272382075133));
#43269=CARTESIAN_POINT('Ctrl Pts',(-20.3015627371329,17.185159703645,-5.71711028276387));
#43270=CARTESIAN_POINT('Ctrl Pts',(-20.3690044710744,17.2411369642621,-5.72149674477641));
#43271=CARTESIAN_POINT('Ctrl Pts',(-20.4324580482224,17.2938040179914,-5.72562381401755));
#43272=CARTESIAN_POINT('Ctrl Pts',(-20.4934979978141,17.3496514870446,-5.72975088325869));
#43273=CARTESIAN_POINT('Ctrl Pts',(-20.5517814829092,17.4084267059583,-5.73387795249984));
#43274=CARTESIAN_POINT('Ctrl Pts',(-20.6102782700972,17.4674170265802,-5.73802012571949));
#43275=CARTESIAN_POINT('Ctrl Pts',(-20.6659979620834,17.5293563204315,-5.74216229893914));
#43276=CARTESIAN_POINT('Ctrl Pts',(-20.7186255971237,17.5939467419898,-5.74630447215879));
#43277=CARTESIAN_POINT('Ctrl Pts',(-20.7709257203662,17.658135205051,-5.75042086784547));
#43278=CARTESIAN_POINT('Ctrl Pts',(-20.8201718394843,17.7249415391099,-5.75453726353214));
#43279=CARTESIAN_POINT('Ctrl Pts',(-20.8660914253506,17.7940362905331,-5.75865365921881));
#43280=CARTESIAN_POINT('Ctrl Pts',(-20.9119829684087,17.8630888462171,-5.76276754104799));
#43281=CARTESIAN_POINT('Ctrl Pts',(-20.9545517475123,17.9344266527042,-5.76688142287717));
#43282=CARTESIAN_POINT('Ctrl Pts',(-20.9935669693931,18.0076891046668,-5.77099530470634));
#43283=CARTESIAN_POINT('Ctrl Pts',(-21.0325708263853,18.0809302157382,-5.77510798818763));
#43284=CARTESIAN_POINT('Ctrl Pts',(-21.0680229592547,18.1560944409463,-5.77922067166891));
#43285=CARTESIAN_POINT('Ctrl Pts',(-21.0997379788824,18.2327956168196,-5.7833333551502));
#43286=CARTESIAN_POINT('Ctrl Pts',(-21.1318415000295,18.3104363640289,-5.78749641803531));
#43287=CARTESIAN_POINT('Ctrl Pts',(-21.1601155043873,18.3896515290328,-5.79165948092042));
#43288=CARTESIAN_POINT('Ctrl Pts',(-21.1844181339266,18.4700202641611,-5.79582254380553));
#43289=CARTESIAN_POINT('Ctrl Pts',(-21.2084475698835,18.5494855487958,-5.79993880837768));
#43290=CARTESIAN_POINT('Ctrl Pts',(-21.2285944016388,18.6300781193823,-5.80405507294983));
#43291=CARTESIAN_POINT('Ctrl Pts',(-21.2447724368935,18.7113783730305,-5.80817133752198));
#43292=CARTESIAN_POINT('Ctrl Pts',(-21.2612263672264,18.7940650953984,-5.81235779956356));
#43293=CARTESIAN_POINT('Ctrl Pts',(-21.2735747867911,18.8774833595966,-5.81654426160515));
#43294=CARTESIAN_POINT('Ctrl Pts',(-21.281781944964,18.9611857471732,-5.82073072364674));
#43295=CARTESIAN_POINT('Ctrl Pts',(-21.2899891031369,19.0448881347499,-5.82491718568833));
#43296=CARTESIAN_POINT('Ctrl Pts',(-21.2940550344004,19.1288741338655,-5.82910364772991));
#43297=CARTESIAN_POINT('Ctrl Pts',(-21.2939994369002,19.2126979607666,-5.8332901097715));
#43298=CARTESIAN_POINT('Ctrl Pts',(-21.2967674808324,19.2126997967162,-5.8332901097715));
#43299=CARTESIAN_POINT('Ctrl Pts',(-21.2975540827487,19.3154768305114,-5.83841759033361));
#43300=CARTESIAN_POINT('Ctrl Pts',(-21.2452321516418,20.267165082075,-5.8859370064562));
#43301=CARTESIAN_POINT('Ctrl Pts',(-20.0538051929683,21.9352257637231,-5.97584835813928));
#43302=CARTESIAN_POINT('Ctrl Pts',(-18.0187465009573,21.8369135205367,-6.06521460546765));
#43303=CARTESIAN_POINT('Ctrl Pts',(-17.2449841467773,21.3000311130452,-6.11218891723554));
#43304=CARTESIAN_POINT('Ctrl Pts',(-17.1725993531626,21.24352550386,-6.11677129344295));
#43305=CARTESIAN_POINT('',(-21.2939992944986,19.2090994299067,-5.76670989019962));
#43306=CARTESIAN_POINT('Ctrl Pts',(-21.293999294499,19.2090994304895,-5.76670989022851));
#43307=CARTESIAN_POINT('Ctrl Pts',(-21.2940618231948,19.2933233519321,-5.77088500205647));
#43308=CARTESIAN_POINT('Ctrl Pts',(-21.2899635861128,19.3775880720651,-5.77506011388443));
#43309=CARTESIAN_POINT('Ctrl Pts',(-21.2817191504239,19.4614538491683,-5.77923522571239));
#43310=CARTESIAN_POINT('Ctrl Pts',(-21.2734754980237,19.5453116583388,-5.78340994087068));
#43311=CARTESIAN_POINT('Ctrl Pts',(-21.2610864747303,19.6287701442277,-5.78758465602897));
#43312=CARTESIAN_POINT('Ctrl Pts',(-21.2446185572459,19.7113943045362,-5.79175937118726));
#43313=CARTESIAN_POINT('Ctrl Pts',(-21.2281473245847,19.794035098017,-5.79593492676264));
#43314=CARTESIAN_POINT('Ctrl Pts',(-21.2075956572653,19.8758407835678,-5.80011048233803));
#43315=CARTESIAN_POINT('Ctrl Pts',(-21.1830809475491,19.956387491411,-5.80428603791341));
#43316=CARTESIAN_POINT('Ctrl Pts',(-21.1585369190256,20.0370305305357,-5.80846658731945));
#43317=CARTESIAN_POINT('Ctrl Pts',(-21.1300205198885,20.1164111473511,-5.8126471367255));
#43318=CARTESIAN_POINT('Ctrl Pts',(-21.0976986239764,20.1941219736187,-5.81682768613154));
#43319=CARTESIAN_POINT('Ctrl Pts',(-21.0653559283573,20.2718828081662,-5.82101092579446));
#43320=CARTESIAN_POINT('Ctrl Pts',(-21.0292030575738,20.347971299817,-5.82519416545738));
#43321=CARTESIAN_POINT('Ctrl Pts',(-20.9894534545796,20.4220035979404,-5.8293774051203));
#43322=CARTESIAN_POINT('Ctrl Pts',(-20.9496320042093,20.4961697093846,-5.83356820598562));
#43323=CARTESIAN_POINT('Ctrl Pts',(-20.906201076148,20.5682718138337,-5.83775900685095));
#43324=CARTESIAN_POINT('Ctrl Pts',(-20.8594180036074,20.6379542073737,-5.84194980771627));
#43325=CARTESIAN_POINT('Ctrl Pts',(-20.8291383592868,20.6830550948788,-5.84466224092617));
#43326=CARTESIAN_POINT('Ctrl Pts',(-20.7974553185202,20.7271429654288,-5.84737467413607));
#43327=CARTESIAN_POINT('Ctrl Pts',(-20.7644472985012,20.770129169764,-5.85008710734597));
#43328=CARTESIAN_POINT('Ctrl Pts',(-20.7135238341689,20.8364465811685,-5.85427174173902));
#43329=CARTESIAN_POINT('Ctrl Pts',(-20.6592531496868,20.9003899294851,-5.85845637613207));
#43330=CARTESIAN_POINT('Ctrl Pts',(-20.6018847443057,20.9616017771012,-5.86264101052512));
#43331=CARTESIAN_POINT('Ctrl Pts',(-20.5445979957491,21.0227264972285,-5.86681968860906));
#43332=CARTESIAN_POINT('Ctrl Pts',(-20.4842225962896,21.0811271065652,-5.87099836669299));
#43333=CARTESIAN_POINT('Ctrl Pts',(-20.4210494366145,21.1364776546142,-5.87517704477693));
#43334=CARTESIAN_POINT('Ctrl Pts',(-20.3567439434538,21.1928203214575,-5.87943062266237));
#43335=CARTESIAN_POINT('Ctrl Pts',(-20.28953969747,21.2460021244011,-5.8836842005478));
#43336=CARTESIAN_POINT('Ctrl Pts',(-20.2197842460679,21.2957170489389,-5.88793777843324));
#43337=CARTESIAN_POINT('Ctrl Pts',(-20.1513811402078,21.3444681526538,-5.89210889241119));
#43338=CARTESIAN_POINT('Ctrl Pts',(-20.0805252582505,21.3898853234968,-5.89628000638915));
#43339=CARTESIAN_POINT('Ctrl Pts',(-20.0075777510545,21.4317205389285,-5.9004511203671));
#43340=CARTESIAN_POINT('Ctrl Pts',(-19.9346547220992,21.4735417161496,-5.90462083468747));
#43341=CARTESIAN_POINT('Ctrl Pts',(-19.8596418605525,21.5117830963985,-5.90879054900784));
#43342=CARTESIAN_POINT('Ctrl Pts',(-19.7829274662089,21.5462411375771,-5.91296026332821));
#43343=CARTESIAN_POINT('Ctrl Pts',(-19.7062158016926,21.5806979525908,-5.91712982927226));
#43344=CARTESIAN_POINT('Ctrl Pts',(-19.6278031447569,21.6113715084927,-5.92129939521631));
#43345=CARTESIAN_POINT('Ctrl Pts',(-19.5480992000003,21.6381057852015,-5.92546896116036));
#43346=CARTESIAN_POINT('Ctrl Pts',(-19.4655929628716,21.6657800060991,-5.92978512389928));
#43347=CARTESIAN_POINT('Ctrl Pts',(-19.3817034451244,21.6892326159303,-5.9341012866382));
#43348=CARTESIAN_POINT('Ctrl Pts',(-19.2969019322697,21.7083468751151,-5.93841744937712));
#43349=CARTESIAN_POINT('Ctrl Pts',(-19.2148628197767,21.7268384893174,-5.9425930135688));
#43350=CARTESIAN_POINT('Ctrl Pts',(-19.1319706883699,21.7412700216399,-5.94676857776048));
#43351=CARTESIAN_POINT('Ctrl Pts',(-19.0486605152119,21.751588270493,-5.95094414195216));
#43352=CARTESIAN_POINT('Ctrl Pts',(-18.9611425432588,21.7624276695664,-5.9553306039647));
#43353=CARTESIAN_POINT('Ctrl Pts',(-18.8731637715282,21.7687272994046,-5.95971706597724));
#43354=CARTESIAN_POINT('Ctrl Pts',(-18.7852297301452,21.7704873538951,-5.96410352798978));
#43355=CARTESIAN_POINT('Ctrl Pts',(-18.6972956887621,21.7722474083857,-5.96848999000232));
#43356=CARTESIAN_POINT('Ctrl Pts',(-18.6094069552492,21.7694679818952,-5.97287645201486));
#43357=CARTESIAN_POINT('Ctrl Pts',(-18.5220617179689,21.7622119011579,-5.97726291402741));
#43358=CARTESIAN_POINT('Ctrl Pts',(-18.4387429644644,21.7552903148049,-5.98144716675325));
#43359=CARTESIAN_POINT('Ctrl Pts',(-18.3556086018994,21.7442699592594,-5.98563141947909));
#43360=CARTESIAN_POINT('Ctrl Pts',(-18.2730941087504,21.7291671428663,-5.98981567220493));
#43361=CARTESIAN_POINT('Ctrl Pts',(-18.190691343858,21.7140847763515,-5.99399425926836));
#43362=CARTESIAN_POINT('Ctrl Pts',(-18.1089072302507,21.6949310074154,-5.99817284633179));
#43363=CARTESIAN_POINT('Ctrl Pts',(-18.0281732667132,21.6717739885202,-6.00235143339522));
#43364=CARTESIAN_POINT('Ctrl Pts',(-17.9475320674686,21.6486435773176,-6.00652521921196));
#43365=CARTESIAN_POINT('Ctrl Pts',(-17.867939059854,21.6215191846037,-6.01069900502871));
#43366=CARTESIAN_POINT('Ctrl Pts',(-17.7898152017479,21.5905199235874,-6.01487279084546));
#43367=CARTESIAN_POINT('Ctrl Pts',(-17.711744863133,21.5595418989095,-6.01904371737058));
#43368=CARTESIAN_POINT('Ctrl Pts',(-17.6351421012572,21.5246944476472,-6.02321464389571));
#43369=CARTESIAN_POINT('Ctrl Pts',(-17.5604112612688,21.4861460331863,-6.02738557042083));
#43370=CARTESIAN_POINT('Ctrl Pts',(-17.4856945971112,21.4476049310452,-6.0315557057552));
#43371=CARTESIAN_POINT('Ctrl Pts',(-17.4128495626245,21.4053644619676,-6.03572584108958));
#43372=CARTESIAN_POINT('Ctrl Pts',(-17.3422580870172,21.3596401391687,-6.03989597642395));
#43373=CARTESIAN_POINT('Ctrl Pts',(-17.284768252093,21.3224021618192,-6.04329214274463));
#43374=CARTESIAN_POINT('Ctrl Pts',(-17.2287727645366,21.2828544582107,-6.04668830906531));
#43375=CARTESIAN_POINT('Ctrl Pts',(-17.1744642439897,21.2411350264762,-6.05008447538598));
#43376=CARTESIAN_POINT('Ctrl Pts',(-17.1744642439897,21.2411350264762,-5.25018233500805));
#43377=CARTESIAN_POINT('Ctrl Pts',(-17.1078623666769,21.1899719226766,-5.2543537667356));
#43378=CARTESIAN_POINT('Ctrl Pts',(-17.0437277229001,21.1354870746848,-5.25852519846314));
#43379=CARTESIAN_POINT('Ctrl Pts',(-16.9824038291382,21.0779522902908,-5.26269663019068));
#43380=CARTESIAN_POINT('Ctrl Pts',(-16.9211032708343,21.0204393994927,-5.26686647457169));
#43381=CARTESIAN_POINT('Ctrl Pts',(-16.8626116736662,20.9598791914874,-5.2710363189527));
#43382=CARTESIAN_POINT('Ctrl Pts',(-16.8072381052118,20.8965825701496,-5.27520616333371));
#43383=CARTESIAN_POINT('Ctrl Pts',(-16.7518689972008,20.8332910474717,-5.27937567182604));
#43384=CARTESIAN_POINT('Ctrl Pts',(-16.6996177211823,20.7672638961413,-5.28354518031838));
#43385=CARTESIAN_POINT('Ctrl Pts',(-16.6507542879591,20.6988465321609,-5.28771468881071));
#43386=CARTESIAN_POINT('Ctrl Pts',(-16.601880133168,20.6304141561077,-5.29188511217262));
#43387=CARTESIAN_POINT('Ctrl Pts',(-16.5563955634883,20.5595909010415,-5.29605553553454));
#43388=CARTESIAN_POINT('Ctrl Pts',(-16.5145275494684,20.4867515594077,-5.30022595889645));
#43389=CARTESIAN_POINT('Ctrl Pts',(-16.4726122570734,20.4138299658258,-5.30440109160139));
#43390=CARTESIAN_POINT('Ctrl Pts',(-16.4343218983041,20.3388881425673,-5.30857622430633));
#43391=CARTESIAN_POINT('Ctrl Pts',(-16.3998374264075,20.2623253920836,-5.31275135701127));
#43392=CARTESIAN_POINT('Ctrl Pts',(-16.3653298664573,20.1857113812853,-5.31692928505226));
#43393=CARTESIAN_POINT('Ctrl Pts',(-16.3346334319057,20.1074747112887,-5.32110721309324));
#43394=CARTESIAN_POINT('Ctrl Pts',(-16.3078800190985,20.0280323361228,-5.32528514113422));
#43395=CARTESIAN_POINT('Ctrl Pts',(-16.2810838876785,19.948463111045,-5.32946974029756));
#43396=CARTESIAN_POINT('Ctrl Pts',(-16.2582434643436,19.867684781143,-5.33365433946089));
#43397=CARTESIAN_POINT('Ctrl Pts',(-16.2394400132345,19.7861264838525,-5.33783893862422));
#43398=CARTESIAN_POINT('Ctrl Pts',(-16.2341302937206,19.7630960475706,-5.33902058595623));
#43399=CARTESIAN_POINT('Ctrl Pts',(-16.2291421595411,19.7400034568201,-5.34020223328824));
#43400=CARTESIAN_POINT('Ctrl Pts',(-16.2244766916358,19.7168584434174,-5.34138388062024));
#43401=CARTESIAN_POINT('Ctrl Pts',(-16.2079546068079,19.634893701071,-5.34556851501329));
#43402=CARTESIAN_POINT('Ctrl Pts',(-16.1954216323759,19.5519661209786,-5.34975314940634));
#43403=CARTESIAN_POINT('Ctrl Pts',(-16.1869832270606,19.4684986570165,-5.35393778379939));
#43404=CARTESIAN_POINT('Ctrl Pts',(-16.1785568327709,19.3851499986583,-5.35811646188333));
#43405=CARTESIAN_POINT('Ctrl Pts',(-16.1742134770096,19.3012634366145,-5.36229513996727));
#43406=CARTESIAN_POINT('Ctrl Pts',(-16.174007684269,19.2172724316078,-5.36647381805121));
#43407=CARTESIAN_POINT('Ctrl Pts',(-16.1737982028414,19.1317759481996,-5.37072739593664));
#43408=CARTESIAN_POINT('Ctrl Pts',(-16.177876170323,19.0461717133522,-5.37498097382208));
#43409=CARTESIAN_POINT('Ctrl Pts',(-16.1862438519479,18.960922791797,-5.37923455170752));
#43410=CARTESIAN_POINT('Ctrl Pts',(-16.1944493097363,18.8773265869357,-5.38340566568547));
#43411=CARTESIAN_POINT('Ctrl Pts',(-16.2067795899915,18.7940725203434,-5.38757677966342));
#43412=CARTESIAN_POINT('Ctrl Pts',(-16.2231843067498,18.7115958004499,-5.39174789364137));
#43413=CARTESIAN_POINT('Ctrl Pts',(-16.2395835187469,18.6291467564162,-5.39591760796175));
#43414=CARTESIAN_POINT('Ctrl Pts',(-16.260054362265,18.5474749918556,-5.40008732228212));
#43415=CARTESIAN_POINT('Ctrl Pts',(-16.2844950829502,18.4670069480508,-5.4042570366025));
#43416=CARTESIAN_POINT('Ctrl Pts',(-16.3089349339296,18.3865417676445,-5.40842660254653));
#43417=CARTESIAN_POINT('Ctrl Pts',(-16.3373442466934,18.3072806627592,-5.41259616849058));
#43418=CARTESIAN_POINT('Ctrl Pts',(-16.3695713807104,18.2296349790806,-5.41676573443461));
#43419=CARTESIAN_POINT('Ctrl Pts',(-16.402931581003,18.14925936895,-5.42108189717353));
#43420=CARTESIAN_POINT('Ctrl Pts',(-16.4403828646776,18.0706153771459,-5.42539805991245));
#43421=CARTESIAN_POINT('Ctrl Pts',(-16.4817035150008,17.9941349525687,-5.42971422265138));
#43422=CARTESIAN_POINT('Ctrl Pts',(-16.5216781494858,17.9201458697778,-5.43388978684306));
#43423=CARTESIAN_POINT('Ctrl Pts',(-16.5652736482194,17.8481819408654,-5.43806535103474));
#43424=CARTESIAN_POINT('Ctrl Pts',(-16.6122442629254,17.7786059926853,-5.44224091522642));
#43425=CARTESIAN_POINT('Ctrl Pts',(-16.6615872517182,17.7055159287637,-5.44662737723896));
#43426=CARTESIAN_POINT('Ctrl Pts',(-16.7146549198489,17.6350618855122,-5.45101383925151));
#43427=CARTESIAN_POINT('Ctrl Pts',(-16.7711149075846,17.5676247799199,-5.45540030126405));
#43428=CARTESIAN_POINT('Ctrl Pts',(-16.8275748953203,17.5001876743276,-5.45978676327659));
#43429=CARTESIAN_POINT('Ctrl Pts',(-16.8874267520075,17.4357678796896,-5.46417322528913));
#43430=CARTESIAN_POINT('Ctrl Pts',(-16.9502957329765,17.3746996193972,-5.46855968730167));
#43431=CARTESIAN_POINT('Ctrl Pts',(-17.010272018937,17.3164412002856,-5.47274432169473));
#43432=CARTESIAN_POINT('Ctrl Pts',(-17.0732171288673,17.2610158259163,-5.47692895608778));
#43433=CARTESIAN_POINT('Ctrl Pts',(-17.1388325082968,17.2087411072957,-5.48111359048083));
#43434=CARTESIAN_POINT('Ctrl Pts',(-17.2043544923552,17.1565407952668,-5.48529226856478));
#43435=CARTESIAN_POINT('Ctrl Pts',(-17.2725388396026,17.1074825154227,-5.48947094664872));
#43436=CARTESIAN_POINT('Ctrl Pts',(-17.3430505912413,17.0618467383004,-5.49364962473267));
#43437=CARTESIAN_POINT('Ctrl Pts',(-17.4148262153522,17.0153929726712,-5.49790320261811));
#43438=CARTESIAN_POINT('Ctrl Pts',(-17.4890131561479,16.9724859492607,-5.50215678050354));
#43439=CARTESIAN_POINT('Ctrl Pts',(-17.5652232755995,16.9333782209288,-5.50641035838897));
#43440=CARTESIAN_POINT('Ctrl Pts',(-17.6399559131736,16.895028672223,-5.51058147236693));
#43441=CARTESIAN_POINT('Ctrl Pts',(-17.716633554776,16.8603326394004,-5.51475258634488));
#43442=CARTESIAN_POINT('Ctrl Pts',(-17.7948629860237,16.8294833259077,-5.51892370032283));
#43443=CARTESIAN_POINT('Ctrl Pts',(-17.8730661666303,16.7986443642001,-5.5230934146432));
#43444=CARTESIAN_POINT('Ctrl Pts',(-17.9528196751248,16.7716497268885,-5.52726312896358));
#43445=CARTESIAN_POINT('Ctrl Pts',(-18.0337098641726,16.7486446792425,-5.53143284328395));
#43446=CARTESIAN_POINT('Ctrl Pts',(-18.1145971748004,16.7256404502148,-5.535602409228));
#43447=CARTESIAN_POINT('Ctrl Pts',(-18.1966206428412,16.7066256536092,-5.53977197517205));
#43448=CARTESIAN_POINT('Ctrl Pts',(-18.2793523115269,16.6916954373546,-5.5439415411161));
#43449=CARTESIAN_POINT('Ctrl Pts',(-18.3649927236227,16.676240293115,-5.54825770385502));
#43450=CARTESIAN_POINT('Ctrl Pts',(-18.4513915445816,16.6651623947289,-5.55257386659394));
#43451=CARTESIAN_POINT('Ctrl Pts',(-18.5380655626732,16.6585091192583,-5.55689002933285));
#43452=CARTESIAN_POINT('Ctrl Pts',(-18.6219161837418,16.6520725735364,-5.56106559352453));
#43453=CARTESIAN_POINT('Ctrl Pts',(-18.7060238760288,16.6497767790178,-5.5652411577162));
#43454=CARTESIAN_POINT('Ctrl Pts',(-18.7899505406878,16.651611491587,-5.56941672190788));
#43455=CARTESIAN_POINT('Ctrl Pts',(-18.8781161416622,16.6535388711264,-5.57380318392041));
#43456=CARTESIAN_POINT('Ctrl Pts',(-18.9660813646938,16.6600249445383,-5.57818964593295));
#43457=CARTESIAN_POINT('Ctrl Pts',(-19.0533460188564,16.670996433026,-5.58257610794549));
#43458=CARTESIAN_POINT('Ctrl Pts',(-19.1406106730191,16.6819679215137,-5.58696256995803));
#43459=CARTESIAN_POINT('Ctrl Pts',(-19.2271742005006,16.6974246482065,-5.59134903197057));
#43460=CARTESIAN_POINT('Ctrl Pts',(-19.3125527301388,16.7172324209243,-5.59573549398311));
#43461=CARTESIAN_POINT('Ctrl Pts',(-19.3940028670669,16.7361288086572,-5.59992012837615));
#43462=CARTESIAN_POINT('Ctrl Pts',(-19.4746778298125,16.7590549809083,-5.60410476276919));
#43463=CARTESIAN_POINT('Ctrl Pts',(-19.5541489559097,16.7859318174286,-5.60828939716224));
#43464=CARTESIAN_POINT('Ctrl Pts',(-19.6335069646957,16.8127703980989,-5.61246807524618));
#43465=CARTESIAN_POINT('Ctrl Pts',(-19.7116641083501,16.8435483273113,-5.61664675333013));
#43466=CARTESIAN_POINT('Ctrl Pts',(-19.7882032486925,16.8781357711075,-5.62082543141408));
#43467=CARTESIAN_POINT('Ctrl Pts',(-19.8661142981178,16.9133431699762,-5.62507900929951));
#43468=CARTESIAN_POINT('Ctrl Pts',(-19.9423482986085,16.9524978888715,-5.62933258718495));
#43469=CARTESIAN_POINT('Ctrl Pts',(-20.0164828014234,16.995410267208,-5.63358616507039));
#43470=CARTESIAN_POINT('Ctrl Pts',(-20.0891800622395,17.0374907053539,-5.63775727904834));
#43471=CARTESIAN_POINT('Ctrl Pts',(-20.15985808817,17.0831841629369,-5.64192839302629));
#43472=CARTESIAN_POINT('Ctrl Pts',(-20.2281415862035,17.1322645862503,-5.64609950700424));
#43473=CARTESIAN_POINT('Ctrl Pts',(-20.2964021710499,17.1813285401536,-5.65026922132462));
#43474=CARTESIAN_POINT('Ctrl Pts',(-20.3622694505382,17.2337769343483,-5.65443893564499));
#43475=CARTESIAN_POINT('Ctrl Pts',(-20.4253973801086,17.289340586222,-5.65860864996537));
#43476=CARTESIAN_POINT('Ctrl Pts',(-20.4885230633163,17.3449022609025,-5.66277821590942));
#43477=CARTESIAN_POINT('Ctrl Pts',(-20.5489092456572,17.4035786682711,-5.66694778185346));
#43478=CARTESIAN_POINT('Ctrl Pts',(-20.6062442778987,17.4650614661805,-5.67111734779751));
#43479=CARTESIAN_POINT('Ctrl Pts',(-20.6655951391432,17.5287059234172,-5.67543351053643));
#43480=CARTESIAN_POINT('Ctrl Pts',(-20.7216759416723,17.5953574026464,-5.67974967327535));
#43481=CARTESIAN_POINT('Ctrl Pts',(-20.7741852955296,17.6646352435778,-5.68406583601427));
#43482=CARTESIAN_POINT('Ctrl Pts',(-20.8249841627081,17.7316563661277,-5.68824140020596));
#43483=CARTESIAN_POINT('Ctrl Pts',(-20.8724404611874,17.8011349549806,-5.69241696439764));
#43484=CARTESIAN_POINT('Ctrl Pts',(-20.9163256700512,17.872697093392,-5.69659252858933));
#43485=CARTESIAN_POINT('Ctrl Pts',(-20.9624274164875,17.9478736652916,-5.70097899060187));
#43486=CARTESIAN_POINT('Ctrl Pts',(-21.004587562026,18.0253492855826,-5.7053654526144));
#43487=CARTESIAN_POINT('Ctrl Pts',(-21.0425969786767,18.1046637084301,-5.70975191462694));
#43488=CARTESIAN_POINT('Ctrl Pts',(-21.0806063953274,18.1839781312776,-5.71413837663948));
#43489=CARTESIAN_POINT('Ctrl Pts',(-21.1144649298774,18.2651307919131,-5.71852483865201));
#43490=CARTESIAN_POINT('Ctrl Pts',(-21.1440235064309,18.3476421955815,-5.72291130066455));
#43491=CARTESIAN_POINT('Ctrl Pts',(-21.1768030234133,18.4391447059575,-5.72777574688617));
#43492=CARTESIAN_POINT('Ctrl Pts',(-21.2043967060816,18.5325974942123,-5.73264019310779));
#43493=CARTESIAN_POINT('Ctrl Pts',(-21.2266026211952,18.6274486545204,-5.73750463932941));
#43494=CARTESIAN_POINT('Ctrl Pts',(-21.2488226674981,18.722360175309,-5.74237218114112));
#43495=CARTESIAN_POINT('Ctrl Pts',(-21.2656479288592,18.818671733481,-5.74723972295282));
#43496=CARTESIAN_POINT('Ctrl Pts',(-21.2769239065508,18.9158085274062,-5.75210726476452));
#43497=CARTESIAN_POINT('Ctrl Pts',(-21.2881998842425,19.0129453213313,-5.75697480657622));
#43498=CARTESIAN_POINT('Ctrl Pts',(-21.2939263955806,19.1109072194806,-5.76184234838792));
#43499=CARTESIAN_POINT('Ctrl Pts',(-21.2939992944986,19.2090994299067,-5.76670989019962));
#43500=CARTESIAN_POINT('Origin',(-18.734,19.211,1.76670989022852));
#43501=CARTESIAN_POINT('',(-17.1718943259277,21.2444859191102,-4.45010592489447));
#43502=CARTESIAN_POINT('',(-17.1769969560721,21.2378276429927,-4.51667469528573));
#43503=CARTESIAN_POINT('',(-17.1744642439897,21.2411350264762,1.76670989022852));
#43504=CARTESIAN_POINT('',(-21.2938494844892,19.2121967450766,-5.03329016024561));
#43505=CARTESIAN_POINT('Ctrl Pts',(-17.1769969560721,21.2378276429927,-4.51667469528573));
#43506=CARTESIAN_POINT('Ctrl Pts',(-16.8552506533971,20.9913954821563,-4.53675462507165));
#43507=CARTESIAN_POINT('Ctrl Pts',(-16.0276177501346,20.0000800476404,-4.59922649041805));
#43508=CARTESIAN_POINT('Ctrl Pts',(-16.1629699362253,17.6131589033056,-4.70409029132493));
#43509=CARTESIAN_POINT('Ctrl Pts',(-18.685881688405,16.1842895105068,-4.83126609800637));
#43510=CARTESIAN_POINT('Ctrl Pts',(-20.9008595855074,17.3473638996065,-4.94099937082188));
#43511=CARTESIAN_POINT('Ctrl Pts',(-21.288210327615,18.7088774717577,-5.00834070807693));
#43512=CARTESIAN_POINT('Ctrl Pts',(-21.2903253369841,19.2121940792196,-5.0332901097715));
#43513=CARTESIAN_POINT('Ctrl Pts',(-21.2939997202205,19.2121968587231,-5.03329016239734));
#43514=CARTESIAN_POINT('Ctrl Pts',(-21.293956476523,19.3046921979846,-5.03786858507676));
#43515=CARTESIAN_POINT('Ctrl Pts',(-21.2888961385951,19.397020737122,-5.04244700775617));
#43516=CARTESIAN_POINT('Ctrl Pts',(-21.2788976615039,19.4886614709891,-5.04702543043559));
#43517=CARTESIAN_POINT('Ctrl Pts',(-21.2688681118718,19.5805869992732,-5.0516180816045));
#43518=CARTESIAN_POINT('Ctrl Pts',(-21.2538698091613,19.6718201549447,-5.0562107327734));
#43519=CARTESIAN_POINT('Ctrl Pts',(-21.234032630531,19.7618510200409,-5.0608033839423));
#43520=CARTESIAN_POINT('Ctrl Pts',(-21.2141037578168,19.8522980379506,-5.06541726388317));
#43521=CARTESIAN_POINT('Ctrl Pts',(-21.1892913049467,19.9415313457699,-5.07003114382404));
#43522=CARTESIAN_POINT('Ctrl Pts',(-21.1597755903685,20.0290542678652,-5.07464502376491));
#43523=CARTESIAN_POINT('Ctrl Pts',(-21.1363775884239,20.0984363421481,-5.07830258629969));
#43524=CARTESIAN_POINT('Ctrl Pts',(-21.1100249393954,20.1667439285117,-5.08196014883446));
#43525=CARTESIAN_POINT('Ctrl Pts',(-21.0808281256645,20.233740313369,-5.08561771136923));
#43526=CARTESIAN_POINT('Ctrl Pts',(-21.0474239145965,20.3103911904541,-5.08980234576228));
#43527=CARTESIAN_POINT('Ctrl Pts',(-21.010198294198,20.3855464442561,-5.09398698015533));
#43528=CARTESIAN_POINT('Ctrl Pts',(-20.9693070771846,20.458798970463,-5.09817161454838));
#43529=CARTESIAN_POINT('Ctrl Pts',(-20.9284740637573,20.5319472307656,-5.10235029263232));
#43530=CARTESIAN_POINT('Ctrl Pts',(-20.8839860396698,20.6031977447538,-5.10652897071627));
#43531=CARTESIAN_POINT('Ctrl Pts',(-20.8360465870689,20.6721639695093,-5.11070764880021));
#43532=CARTESIAN_POINT('Ctrl Pts',(-20.7872478542335,20.7423663642784,-5.11496122668564));
#43533=CARTESIAN_POINT('Ctrl Pts',(-20.734872934752,20.8102013305707,-5.11921480457108));
#43534=CARTESIAN_POINT('Ctrl Pts',(-20.6791852047648,20.8752879916541,-5.12346838245652));
#43535=CARTESIAN_POINT('Ctrl Pts',(-20.6245770900892,20.9391128208061,-5.12763949643447));
#43536=CARTESIAN_POINT('Ctrl Pts',(-20.5667837820758,21.0002945906742,-5.13181061041242));
#43537=CARTESIAN_POINT('Ctrl Pts',(-20.506095860174,21.0585054160554,-5.13598172439037));
#43538=CARTESIAN_POINT('Ctrl Pts',(-20.4454283026906,21.1166967082319,-5.14015143871074));
#43539=CARTESIAN_POINT('Ctrl Pts',(-20.381868392088,21.1719187176573,-5.14432115303111));
#43540=CARTESIAN_POINT('Ctrl Pts',(-20.3157437934275,21.2238801683045,-5.14849086735148));
#43541=CARTESIAN_POINT('Ctrl Pts',(-20.249621547764,21.2758397699403,-5.15266043329553));
#43542=CARTESIAN_POINT('Ctrl Pts',(-20.1809351577379,21.324538759915,-5.15682999923957));
#43543=CARTESIAN_POINT('Ctrl Pts',(-20.1100445342431,21.3697268098997,-5.16099956518362));
#43544=CARTESIAN_POINT('Ctrl Pts',(-20.0366614838793,21.4165036159763,-5.16531572792254));
#43545=CARTESIAN_POINT('Ctrl Pts',(-19.9609167591476,21.4595177156539,-5.16963189066146));
#43546=CARTESIAN_POINT('Ctrl Pts',(-19.8832395142305,21.4985420299813,-5.17394805340038));
#43547=CARTESIAN_POINT('Ctrl Pts',(-19.8080925973964,21.5362951313742,-5.17812361759206));
#43548=CARTESIAN_POINT('Ctrl Pts',(-19.7311375805023,21.5703142429022,-5.18229918178374));
#43549=CARTESIAN_POINT('Ctrl Pts',(-19.6527837251098,21.6004427104397,-5.18647474597542));
#43550=CARTESIAN_POINT('Ctrl Pts',(-19.5704724027501,21.6320928952489,-5.19086120798796));
#43551=CARTESIAN_POINT('Ctrl Pts',(-19.4866177726056,21.6594488930308,-5.1952476700005));
#43552=CARTESIAN_POINT('Ctrl Pts',(-19.401710454222,21.6823888300554,-5.19963413201304));
#43553=CARTESIAN_POINT('Ctrl Pts',(-19.3168031358385,21.7053287670799,-5.20402059402559));
#43554=CARTESIAN_POINT('Ctrl Pts',(-19.2308437124363,21.723852595477,-5.20840705603813));
#43555=CARTESIAN_POINT('Ctrl Pts',(-19.1443308019265,21.7379009939035,-5.21279351805067));
#43556=CARTESIAN_POINT('Ctrl Pts',(-19.0590101810525,21.7517557823849,-5.2171195274306));
#43557=CARTESIAN_POINT('Ctrl Pts',(-18.9728228912871,21.7613111055906,-5.22144553681052));
#43558=CARTESIAN_POINT('Ctrl Pts',(-18.8862405443866,21.7664691969665,-5.22577154619045));
#43559=CARTESIAN_POINT('Ctrl Pts',(-18.8026253778788,21.7714505203506,-5.22994930306083));
#43560=CARTESIAN_POINT('Ctrl Pts',(-18.7186422980839,21.7723310237495,-5.2341270599312));
#43561=CARTESIAN_POINT('Ctrl Pts',(-18.6347264664641,21.7690744253323,-5.23830481680158));
#43562=CARTESIAN_POINT('Ctrl Pts',(-18.5508928335468,21.7658210168754,-5.24247848140252));
#43563=CARTESIAN_POINT('Ctrl Pts',(-18.4671267750382,21.7584385707795,-5.24665214600345));
#43564=CARTESIAN_POINT('Ctrl Pts',(-18.3838655165602,21.7469427918441,-5.25082581060438));
#43565=CARTESIAN_POINT('Ctrl Pts',(-18.3006608358562,21.735454824532,-5.25499663911255));
#43566=CARTESIAN_POINT('Ctrl Pts',(-18.217960728171,21.7198591392685,-5.25916746762072));
#43567=CARTESIAN_POINT('Ctrl Pts',(-18.1361979890339,21.7002233237869,-5.26333829612888));
#43568=CARTESIAN_POINT('Ctrl Pts',(-18.0544662814438,21.6805949607188,-5.26750754167564));
#43569=CARTESIAN_POINT('Ctrl Pts',(-17.9736716819021,21.6569296230204,-5.27167678722239));
#43570=CARTESIAN_POINT('Ctrl Pts',(-17.894236126945,21.6293458473741,-5.27584603276915));
#43571=CARTESIAN_POINT('Ctrl Pts',(-17.8147812397687,21.6017553586685,-5.28001629298458));
#43572=CARTESIAN_POINT('Ctrl Pts',(-17.7366864944959,21.5702446726599,-5.28418655320001));
#43573=CARTESIAN_POINT('Ctrl Pts',(-17.6603571013659,21.5349816966174,-5.28835681341544));
#43574=CARTESIAN_POINT('Ctrl Pts',(-17.5840157675873,21.4997132041835,-5.29252772600881));
#43575=CARTESIAN_POINT('Ctrl Pts',(-17.5094407480921,21.4606914573206,-5.29669863860218));
#43576=CARTESIAN_POINT('Ctrl Pts',(-17.4370140541151,21.418131046444,-5.30086955119554));
#43577=CARTESIAN_POINT('Ctrl Pts',(-17.3645257193928,21.3755344133502,-5.30504401355968));
#43578=CARTESIAN_POINT('Ctrl Pts',(-17.294189747792,21.3293933517496,-5.30921847592382));
#43579=CARTESIAN_POINT('Ctrl Pts',(-17.2263597646639,21.2799661478129,-5.31339293828795));
#43580=CARTESIAN_POINT('Ctrl Pts',(-17.2088933668714,21.2672385137208,-5.31446787324827));
#43581=CARTESIAN_POINT('Ctrl Pts',(-17.1915929675281,21.254293194019,-5.31554280820858));
#43582=CARTESIAN_POINT('Ctrl Pts',(-17.1744642439897,21.2411350264762,-5.31661774316889));
#43583=CARTESIAN_POINT('',(-21.2942631007509,19.2101644346482,-4.96670989022851));
#43584=CARTESIAN_POINT('Ctrl Pts',(-21.2939998636668,19.210164520558,-4.96670989022851));
#43585=CARTESIAN_POINT('Ctrl Pts',(-21.2940269378475,19.2931227545131,-4.97085977152528));
#43586=CARTESIAN_POINT('Ctrl Pts',(-21.2900172964774,19.3762448671897,-4.97500965282206));
#43587=CARTESIAN_POINT('Ctrl Pts',(-21.2819493183893,19.4591013319584,-4.97915953411883));
#43588=CARTESIAN_POINT('Ctrl Pts',(-21.273892503302,19.5418431550195,-4.98330367356457));
#43589=CARTESIAN_POINT('Ctrl Pts',(-21.2617885455564,19.6243195978693,-4.9874478130103));
#43590=CARTESIAN_POINT('Ctrl Pts',(-21.2456678375727,19.7061006702713,-4.99159195245604));
#43591=CARTESIAN_POINT('Ctrl Pts',(-21.2295645603718,19.787793315532,-4.99573161098226));
#43592=CARTESIAN_POINT('Ctrl Pts',(-21.2094532518121,19.8687916269892,-4.99987126950847));
#43593=CARTESIAN_POINT('Ctrl Pts',(-21.185415992005,19.9486717658566,-5.00401092803468));
#43594=CARTESIAN_POINT('Ctrl Pts',(-21.1613926712712,20.0285055826756,-5.00814818599593));
#43595=CARTESIAN_POINT('Ctrl Pts',(-21.1334480518402,20.1072220663071,-5.01228544395718));
#43596=CARTESIAN_POINT('Ctrl Pts',(-21.1017147974227,20.1844097996556,-5.01642270191842));
#43597=CARTESIAN_POINT('Ctrl Pts',(-21.0699900384709,20.2615768686961,-5.02055885227398));
#43598=CARTESIAN_POINT('Ctrl Pts',(-21.0344788364884,20.3372155671953,-5.02469500262954));
#43599=CARTESIAN_POINT('Ctrl Pts',(-20.9953624823965,20.4109332161455,-5.02883115298509));
#43600=CARTESIAN_POINT('Ctrl Pts',(-20.9562443890678,20.4846541428155,-5.03296748724698));
#43601=CARTESIAN_POINT('Ctrl Pts',(-20.9135210465748,20.5564534375451,-5.03710382150886));
#43602=CARTESIAN_POINT('Ctrl Pts',(-20.8674196102005,20.6259631680054,-5.04124015577075));
#43603=CARTESIAN_POINT('Ctrl Pts',(-20.8212714994521,20.6955432720466,-5.04538067777227));
#43604=CARTESIAN_POINT('Ctrl Pts',(-20.7717387262307,20.7628287929985,-5.0495211997738));
#43605=CARTESIAN_POINT('Ctrl Pts',(-20.7190913321275,20.8274814886389,-5.05366172177532));
#43606=CARTESIAN_POINT('Ctrl Pts',(-20.6664157771977,20.8921687666814,-5.05780445852126));
#43607=CARTESIAN_POINT('Ctrl Pts',(-20.6106225991445,20.9542200685987,-5.0619471952672));
#43608=CARTESIAN_POINT('Ctrl Pts',(-20.5520199344765,21.0133327988598,-5.06608993201314));
#43609=CARTESIAN_POINT('Ctrl Pts',(-20.4933173061603,21.0725463628324,-5.07023973538449));
#43610=CARTESIAN_POINT('Ctrl Pts',(-20.4317959684764,21.1288110311776,-5.07438953875584));
#43611=CARTESIAN_POINT('Ctrl Pts',(-20.3677981562815,21.181863664623,-5.07853934212718));
#43612=CARTESIAN_POINT('Ctrl Pts',(-20.3241391698325,21.218055905033,-5.08137031717058));
#43613=CARTESIAN_POINT('Ctrl Pts',(-20.2793283343472,21.252754156268,-5.08420129221397));
#43614=CARTESIAN_POINT('Ctrl Pts',(-20.2334815623284,21.2858867545572,-5.08703226725737));
#43615=CARTESIAN_POINT('Ctrl Pts',(-20.165712692572,21.3348620398235,-5.09121690165042));
#43616=CARTESIAN_POINT('Ctrl Pts',(-20.0954157767524,21.38060482739,-5.09540153604347));
#43617=CARTESIAN_POINT('Ctrl Pts',(-20.0229321512534,21.4228440065848,-5.09958617043652));
#43618=CARTESIAN_POINT('Ctrl Pts',(-19.9505516972235,21.4650230635363,-5.10376484852047));
#43619=CARTESIAN_POINT('Ctrl Pts',(-19.875991110009,21.5037081881332,-5.10794352660443));
#43620=CARTESIAN_POINT('Ctrl Pts',(-19.7996223782739,21.5386702831204,-5.11212220468838));
#43621=CARTESIAN_POINT('Ctrl Pts',(-19.7218847919078,21.5742590485334,-5.11637578257381));
#43622=CARTESIAN_POINT('Ctrl Pts',(-19.642273992229,21.6059897185087,-5.12062936045925));
#43623=CARTESIAN_POINT('Ctrl Pts',(-19.5612105522304,21.6336685085415,-5.12488293834468));
#43624=CARTESIAN_POINT('Ctrl Pts',(-19.4817186851983,21.6608106912188,-5.12905405232263));
#43625=CARTESIAN_POINT('Ctrl Pts',(-19.4008304551544,21.6840565436591,-5.13322516630058));
#43626=CARTESIAN_POINT('Ctrl Pts',(-19.3189628776791,21.7032717411505,-5.13739628027853));
#43627=CARTESIAN_POINT('Ctrl Pts',(-19.2371227716599,21.7224804907969,-5.14156599459891));
#43628=CARTESIAN_POINT('Ctrl Pts',(-19.1543044183623,21.7376611666004,-5.14573570891929));
#43629=CARTESIAN_POINT('Ctrl Pts',(-19.0709381209922,21.7487298324728,-5.14990542323966));
#43630=CARTESIAN_POINT('Ctrl Pts',(-18.9875747901529,21.7597981044745,-5.15407498918371));
#43631=CARTESIAN_POINT('Ctrl Pts',(-18.9036640101517,21.7667545977695,-5.15824455512775));
#43632=CARTESIAN_POINT('Ctrl Pts',(-18.819642997584,21.7695670358552,-5.16241412107179));
#43633=CARTESIAN_POINT('Ctrl Pts',(-18.7326679098656,21.7724783557944,-5.16673028381071));
#43634=CARTESIAN_POINT('Ctrl Pts',(-18.6455752209303,21.7709487709587,-5.17104644654963));
#43635=CARTESIAN_POINT('Ctrl Pts',(-18.5588499153533,21.7650012623036,-5.17536260928855));
#43636=CARTESIAN_POINT('Ctrl Pts',(-18.4749496774835,21.7592474931173,-5.17953817348023));
#43637=CARTESIAN_POINT('Ctrl Pts',(-18.3913937177404,21.749359309981,-5.18371373767191));
#43638=CARTESIAN_POINT('Ctrl Pts',(-18.3086140512033,21.7354101874629,-5.18788930186359));
#43639=CARTESIAN_POINT('Ctrl Pts',(-18.2216533804995,21.7207565279272,-5.19227576387613));
#43640=CARTESIAN_POINT('Ctrl Pts',(-18.1355500550633,21.701621038382,-5.19666222588866));
#43641=CARTESIAN_POINT('Ctrl Pts',(-18.0507884164764,21.6781485427795,-5.2010486879012));
#43642=CARTESIAN_POINT('Ctrl Pts',(-17.9660267778894,21.654676047177,-5.20543514991373));
#43643=CARTESIAN_POINT('Ctrl Pts',(-17.8826073525323,21.6268668011753,-5.20982161192627));
#43644=CARTESIAN_POINT('Ctrl Pts',(-17.8009895271363,21.5949235427183,-5.21420807393881));
#43645=CARTESIAN_POINT('Ctrl Pts',(-17.723133526371,21.5644525721575,-5.21839236074317));
#43646=CARTESIAN_POINT('Ctrl Pts',(-17.6466269368319,21.5301068697023,-5.22257664754754));
#43647=CARTESIAN_POINT('Ctrl Pts',(-17.5718823763611,21.4920266611392,-5.2267609343519));
#43648=CARTESIAN_POINT('Ctrl Pts',(-17.497252122809,21.4540046886708,-5.23093882212296));
#43649=CARTESIAN_POINT('Ctrl Pts',(-17.4243789496118,21.4122597663377,-5.23511670989402));
#43650=CARTESIAN_POINT('Ctrl Pts',(-17.3536566218709,21.3669805561403,-5.23929459766508));
#43651=CARTESIAN_POINT('Ctrl Pts',(-17.2922215801368,21.327647430987,-5.24292384344607));
#43652=CARTESIAN_POINT('Ctrl Pts',(-17.2324094767135,21.2856481554772,-5.24655308922706));
#43653=CARTESIAN_POINT('Ctrl Pts',(-17.1744642439897,21.2411350264762,-5.25018233500805));
#43654=CARTESIAN_POINT('Ctrl Pts',(-17.1718943259273,21.2444859191099,-4.45010592489449));
#43655=CARTESIAN_POINT('Ctrl Pts',(-17.1663500721053,21.2402338685243,-4.45045502787973));
#43656=CARTESIAN_POINT('Ctrl Pts',(-16.4898974816279,20.7166175504919,-4.49319606642544));
#43657=CARTESIAN_POINT('Ctrl Pts',(-15.7195027796251,18.9351410654681,-4.57832904053163));
#43658=CARTESIAN_POINT('Ctrl Pts',(-17.3342635373914,16.5269676830084,-4.70550484721307));
#43659=CARTESIAN_POINT('Ctrl Pts',(-20.2331956221585,16.5812273615557,-4.8326806538945));
#43660=CARTESIAN_POINT('Ctrl Pts',(-21.2762381336493,18.2701494254144,-4.91974900156631));
#43661=CARTESIAN_POINT('Ctrl Pts',(-21.2980949765117,19.1644257538227,-4.96442541367765));
#43662=CARTESIAN_POINT('Ctrl Pts',(-21.2979002687903,19.210163247625,-4.96670989022851));
#43663=CARTESIAN_POINT('Origin',(-18.734,19.211,1.76670989022852));
#43664=CARTESIAN_POINT('',(-17.1744642439897,21.2411350264762,-3.6500459524789));
#43665=CARTESIAN_POINT('',(-17.1744642439897,21.2411350264762,-3.71676814526475));
#43666=CARTESIAN_POINT('',(-17.1744642439897,21.2411350264762,1.76670989022852));
#43667=CARTESIAN_POINT('',(-21.2939990418858,19.2087851537695,-4.23329008725203));
#43668=CARTESIAN_POINT('Ctrl Pts',(-17.1744642439897,21.2411350264762,-3.71676814526475));
#43669=CARTESIAN_POINT('Ctrl Pts',(-17.1078988246138,21.1899999294128,-3.72094075707419));
#43670=CARTESIAN_POINT('Ctrl Pts',(-17.0437864698061,21.1355379119879,-3.72511336888363));
#43671=CARTESIAN_POINT('Ctrl Pts',(-16.9824731010997,21.0780172796277,-3.72928598069307));
#43672=CARTESIAN_POINT('Ctrl Pts',(-16.9211917165634,21.0205266529536,-3.73345641585606));
#43673=CARTESIAN_POINT('Ctrl Pts',(-16.8627067539701,20.9599808934146,-3.73762685101905));
#43674=CARTESIAN_POINT('Ctrl Pts',(-16.8073301828919,20.8966878168405,-3.74179728618204));
#43675=CARTESIAN_POINT('Ctrl Pts',(-16.7519658872628,20.8334087705851,-3.74596679687528));
#43676=CARTESIAN_POINT('Ctrl Pts',(-16.6997089170967,20.7673839632324,-3.75013630756853));
#43677=CARTESIAN_POINT('Ctrl Pts',(-16.6508326185409,20.6989562025896,-3.75430581826177));
#43678=CARTESIAN_POINT('Ctrl Pts',(-16.6019524929159,20.630523083976,-3.75847565543239));
#43679=CARTESIAN_POINT('Ctrl Pts',(-16.5564538308376,20.5596870135816,-3.76264549260301));
#43680=CARTESIAN_POINT('Ctrl Pts',(-16.5145672996359,20.4868207117594,-3.76681532977363));
#43681=CARTESIAN_POINT('Ctrl Pts',(-16.4726368702626,20.4138780441624,-3.77098953704179));
#43682=CARTESIAN_POINT('Ctrl Pts',(-16.4343263606549,20.3389012961015,-3.77516374430996));
#43683=CARTESIAN_POINT('Ctrl Pts',(-16.3998207425502,20.262288349641,-3.77933795157812));
#43684=CARTESIAN_POINT('Ctrl Pts',(-16.365296388734,20.1856338042138,-3.78351442533932));
#43685=CARTESIAN_POINT('Ctrl Pts',(-16.3345812083815,20.1073417197765,-3.78769089910052));
#43686=CARTESIAN_POINT('Ctrl Pts',(-16.3078113066412,20.0278282709468,-3.79186737286172));
#43687=CARTESIAN_POINT('Ctrl Pts',(-16.2809949059668,19.9481767084005,-3.79605110109774));
#43688=CARTESIAN_POINT('Ctrl Pts',(-16.2581375967678,19.8672999871918,-3.80023482933376));
#43689=CARTESIAN_POINT('Ctrl Pts',(-16.2393250174113,19.7856274717117,-3.80441855756978));
#43690=CARTESIAN_POINT('Ctrl Pts',(-16.2251740665448,19.7241928469432,-3.80756558656482));
#43691=CARTESIAN_POINT('Ctrl Pts',(-16.2133106294126,19.6623082203732,-3.81071261555985));
#43692=CARTESIAN_POINT('Ctrl Pts',(-16.2037517912764,19.6001580684646,-3.81385964455489));
#43693=CARTESIAN_POINT('Ctrl Pts',(-16.1910413132713,19.5175164202231,-3.81804427894799));
#43694=CARTESIAN_POINT('Ctrl Pts',(-16.182360236898,19.4340976099864,-3.8222289133411));
#43695=CARTESIAN_POINT('Ctrl Pts',(-16.1777943305988,19.3503290196653,-3.8264135477342));
#43696=CARTESIAN_POINT('Ctrl Pts',(-16.1732349233019,19.266679663564,-3.8305922258182));
#43697=CARTESIAN_POINT('Ctrl Pts',(-16.1727790761929,19.1826819717243,-3.8347709039022));
#43698=CARTESIAN_POINT('Ctrl Pts',(-16.1764611917473,19.0987714640513,-3.8389495819862));
#43699=CARTESIAN_POINT('Ctrl Pts',(-16.1802093065766,19.0133569208352,-3.84320315987162));
#43700=CARTESIAN_POINT('Ctrl Pts',(-16.1882452624471,18.9280331946169,-3.84745673775704));
#43701=CARTESIAN_POINT('Ctrl Pts',(-16.2005498883094,18.8432629586585,-3.85171031564246));
#43702=CARTESIAN_POINT('Ctrl Pts',(-16.212615964989,18.7601361591384,-3.85588142962047));
#43703=CARTESIAN_POINT('Ctrl Pts',(-16.2287866065491,18.6775420566428,-3.86005254359848));
#43704=CARTESIAN_POINT('Ctrl Pts',(-16.2489913365583,18.5959130609259,-3.86422365757649));
#43705=CARTESIAN_POINT('Ctrl Pts',(-16.2691892866751,18.5143114566068,-3.86839337189693));
#43706=CARTESIAN_POINT('Ctrl Pts',(-16.293418526377,18.4336747620786,-3.87256308621736));
#43707=CARTESIAN_POINT('Ctrl Pts',(-16.3215576717042,18.3544242516587,-3.87673280053779));
#43708=CARTESIAN_POINT('Ctrl Pts',(-16.3496958157198,18.275176561312,-3.8809023664819));
#43709=CARTESIAN_POINT('Ctrl Pts',(-16.3817434340021,18.1973153902317,-3.885071932426));
#43710=CARTESIAN_POINT('Ctrl Pts',(-16.4175300086123,18.1212446242388,-3.88924149837011));
#43711=CARTESIAN_POINT('Ctrl Pts',(-16.4545747950371,18.0424993039595,-3.89355766110896));
#43712=CARTESIAN_POINT('Ctrl Pts',(-16.4956261286209,17.9656731098166,-3.89787382384781));
#43713=CARTESIAN_POINT('Ctrl Pts',(-16.5404425366712,17.8911872651491,-3.90218998658667));
#43714=CARTESIAN_POINT('Ctrl Pts',(-16.5837990549445,17.8191277890349,-3.9063655507784));
#43715=CARTESIAN_POINT('Ctrl Pts',(-16.6306788183653,17.7492588949824,-3.91054111497015));
#43716=CARTESIAN_POINT('Ctrl Pts',(-16.6808195479048,17.681931646023,-3.91471667916188));
#43717=CARTESIAN_POINT('Ctrl Pts',(-16.7334927664927,17.6112038577771,-3.91910314117429));
#43718=CARTESIAN_POINT('Ctrl Pts',(-16.789764658884,17.5432816689319,-3.9234896031867));
#43719=CARTESIAN_POINT('Ctrl Pts',(-16.8492855900871,17.4785302042844,-3.92787606519911));
#43720=CARTESIAN_POINT('Ctrl Pts',(-16.9088065212903,17.413778739637,-3.93226252721152));
#43721=CARTESIAN_POINT('Ctrl Pts',(-16.9715760238564,17.3521983512228,-3.93664898922392));
#43722=CARTESIAN_POINT('Ctrl Pts',(-17.0372042845901,17.2941055584184,-3.94103545123633));
#43723=CARTESIAN_POINT('Ctrl Pts',(-17.0998128917648,17.2386857011235,-3.94522008562937));
#43724=CARTESIAN_POINT('Ctrl Pts',(-17.1652560078683,17.1862332698863,-3.9494047200224));
#43725=CARTESIAN_POINT('Ctrl Pts',(-17.2332206971797,17.1370517161158,-3.95358935441543));
#43726=CARTESIAN_POINT('Ctrl Pts',(-17.3010886471682,17.0879401661996,-3.95776803249936));
#43727=CARTESIAN_POINT('Ctrl Pts',(-17.3714706716869,17.0420905134701,-3.96194671058329));
#43728=CARTESIAN_POINT('Ctrl Pts',(-17.4440191888255,16.9997674236297,-3.96612538866722));
#43729=CARTESIAN_POINT('Ctrl Pts',(-17.5178680859944,16.9566857228207,-3.97037896655266));
#43730=CARTESIAN_POINT('Ctrl Pts',(-17.5939615474704,16.9172585752801,-3.9746325444381));
#43731=CARTESIAN_POINT('Ctrl Pts',(-17.6719001613345,16.881720297451,-3.97888612232354));
#43732=CARTESIAN_POINT('Ctrl Pts',(-17.7483277830838,16.846870998485,-3.98305723630147));
#43733=CARTESIAN_POINT('Ctrl Pts',(-17.8265292140571,16.815761327818,-3.98722835027941));
#43734=CARTESIAN_POINT('Ctrl Pts',(-17.9061027185259,16.7885660811226,-3.99139946425735));
#43735=CARTESIAN_POINT('Ctrl Pts',(-17.9856495213366,16.761379960055,-3.9955691785777));
#43736=CARTESIAN_POINT('Ctrl Pts',(-18.0665670483063,16.7381058029316,-3.99973889289804));
#43737=CARTESIAN_POINT('Ctrl Pts',(-18.1484353715671,16.7188695728497,-4.00390860721839));
#43738=CARTESIAN_POINT('Ctrl Pts',(-18.2303007816016,16.6996340272755,-4.00807817316241));
#43739=CARTESIAN_POINT('Ctrl Pts',(-18.313116472626,16.6844362274532,-4.01224773910643));
#43740=CARTESIAN_POINT('Ctrl Pts',(-18.3964505424551,16.6733514105158,-4.01641730505044));
#43741=CARTESIAN_POINT('Ctrl Pts',(-18.4827145353766,16.6618768650894,-4.02073346778938));
#43742=CARTESIAN_POINT('Ctrl Pts',(-18.5695335149127,16.6548099783526,-4.02504963052833));
#43743=CARTESIAN_POINT('Ctrl Pts',(-18.6564225943068,16.6521757101892,-4.02936579326727));
#43744=CARTESIAN_POINT('Ctrl Pts',(-18.7404812710779,16.6496272530341,-4.03354135745893));
#43745=CARTESIAN_POINT('Ctrl Pts',(-18.8246050807771,16.6512270080048,-4.03771692165059));
#43746=CARTESIAN_POINT('Ctrl Pts',(-18.9083568682879,16.6569444637047,-4.04189248584225));
#43747=CARTESIAN_POINT('Ctrl Pts',(-18.9963387594864,16.6629506945001,-4.04627894785483));
#43748=CARTESIAN_POINT('Ctrl Pts',(-19.08390947946,16.6735014582054,-4.05066540986742));
#43749=CARTESIAN_POINT('Ctrl Pts',(-19.1705727652473,16.6885004022509,-4.05505187188));
#43750=CARTESIAN_POINT('Ctrl Pts',(-19.2572360510346,16.7034993462965,-4.05943833389259));
#43751=CARTESIAN_POINT('Ctrl Pts',(-19.342991353608,16.7229462681819,-4.06382479590517));
#43752=CARTESIAN_POINT('Ctrl Pts',(-19.4273615317729,16.7466847226344,-4.06821125791776));
#43753=CARTESIAN_POINT('Ctrl Pts',(-19.5078497129729,16.7693309356085,-4.0723958923108));
#43754=CARTESIAN_POINT('Ctrl Pts',(-19.5873770243864,16.7959667334644,-4.07658052670384));
#43755=CARTESIAN_POINT('Ctrl Pts',(-19.6655189252299,16.826493239276,-4.08076516109689));
#43756=CARTESIAN_POINT('Ctrl Pts',(-19.7435496007498,16.8569762943851,-4.08494383918084));
#43757=CARTESIAN_POINT('Ctrl Pts',(-19.8201983578021,16.8913388913937,-4.08912251726478));
#43758=CARTESIAN_POINT('Ctrl Pts',(-19.8950545149197,16.9294320274459,-4.09330119534873));
#43759=CARTESIAN_POINT('Ctrl Pts',(-19.9712524148554,16.9682079555848,-4.09755477323417));
#43760=CARTESIAN_POINT('Ctrl Pts',(-20.0455923539259,17.0108493474662,-4.1018083511196));
#43761=CARTESIAN_POINT('Ctrl Pts',(-20.1176611149876,17.0571471919207,-4.10606192900504));
#43762=CARTESIAN_POINT('Ctrl Pts',(-20.1883326824854,17.1025474623176,-4.11023304298298));
#43763=CARTESIAN_POINT('Ctrl Pts',(-20.2568199436827,17.1514634154309,-4.11440415696093));
#43764=CARTESIAN_POINT('Ctrl Pts',(-20.3227584711506,17.2036518686717,-4.11857527093887));
#43765=CARTESIAN_POINT('Ctrl Pts',(-20.3886748723087,17.2558228095729,-4.12274498525924));
#43766=CARTESIAN_POINT('Ctrl Pts',(-20.4520438778608,17.3112637844568,-4.1269146995796));
#43767=CARTESIAN_POINT('Ctrl Pts',(-20.5125322737859,17.369689881877,-4.13108441389996));
#43768=CARTESIAN_POINT('Ctrl Pts',(-20.5730185172743,17.4281139002461,-4.135253979844));
#43769=CARTESIAN_POINT('Ctrl Pts',(-20.6306240246489,17.489522509736,-4.13942354578804));
#43770=CARTESIAN_POINT('Ctrl Pts',(-20.6850517529259,17.5535932733922,-4.14359311173208));
#43771=CARTESIAN_POINT('Ctrl Pts',(-20.7413930929854,17.6199166860588,-4.14790927447101));
#43772=CARTESIAN_POINT('Ctrl Pts',(-20.7943286933423,17.6890925366906,-4.15222543720993));
#43773=CARTESIAN_POINT('Ctrl Pts',(-20.8435751066798,17.7607266225719,-4.15654159994886));
#43774=CARTESIAN_POINT('Ctrl Pts',(-20.8912173232825,17.83002723564,-4.16071716414053));
#43775=CARTESIAN_POINT('Ctrl Pts',(-20.9354068051749,17.9016279637396,-4.16489272833221));
#43776=CARTESIAN_POINT('Ctrl Pts',(-20.9759325838396,17.9751447133591,-4.16906829252388));
#43777=CARTESIAN_POINT('Ctrl Pts',(-21.018505223244,18.0523746192327,-4.17345475453643));
#43778=CARTESIAN_POINT('Ctrl Pts',(-21.0570340704737,18.1317186646457,-4.17784121654899));
#43779=CARTESIAN_POINT('Ctrl Pts',(-21.0913315250629,18.2127074171643,-4.18222767856154));
#43780=CARTESIAN_POINT('Ctrl Pts',(-21.125628979652,18.2936961696829,-4.18661414057409));
#43781=CARTESIAN_POINT('Ctrl Pts',(-21.1556949146933,18.3763290580522,-4.19100060258664));
#43782=CARTESIAN_POINT('Ctrl Pts',(-21.1814026084241,18.4601202011779,-4.19538706459919));
#43783=CARTESIAN_POINT('Ctrl Pts',(-21.211365847261,18.557781782967,-4.20049964335899));
#43784=CARTESIAN_POINT('Ctrl Pts',(-21.2355013786602,18.6573099274653,-4.20561222211879));
#43785=CARTESIAN_POINT('Ctrl Pts',(-21.2536149670824,18.758075704279,-4.21072480087859));
#43786=CARTESIAN_POINT('Ctrl Pts',(-21.271481685507,18.8574681448711,-4.2157677003304));
#43787=CARTESIAN_POINT('Ctrl Pts',(-21.2834894543748,18.9580647258708,-4.22081059978222));
#43788=CARTESIAN_POINT('Ctrl Pts',(-21.289497836736,19.0592409592887,-4.22585349923404));
#43789=CARTESIAN_POINT('Ctrl Pts',(-21.2924512874047,19.1089746473736,-4.2283323619067));
#43790=CARTESIAN_POINT('Ctrl Pts',(-21.293955837589,19.1588480714825,-4.23081122457936));
#43791=CARTESIAN_POINT('Ctrl Pts',(-21.2939990418858,19.2087851537695,-4.23329008725203));
#43792=CARTESIAN_POINT('Ctrl Pts',(-21.2923873880696,19.2087870015046,-4.2332901097715));
#43793=CARTESIAN_POINT('Ctrl Pts',(-21.2874613882922,19.8078856368616,-4.26304769694121));
#43794=CARTESIAN_POINT('Ctrl Pts',(-20.7784814085672,21.2679844548948,-4.3351972196714));
#43795=CARTESIAN_POINT('Ctrl Pts',(-18.7708037338048,22.0472233474103,-4.42965874817614));
#43796=CARTESIAN_POINT('Ctrl Pts',(-17.5345084334408,21.5116530922966,-4.49436268951118));
#43797=CARTESIAN_POINT('Ctrl Pts',(-17.1769969560721,21.2378276429927,-4.51667469528573));
#43798=CARTESIAN_POINT('',(-21.2939989159607,19.2133559031925,-4.16670989022851));
#43799=CARTESIAN_POINT('Ctrl Pts',(-21.2939117877142,19.2133565885178,-4.16670992830965));
#43800=CARTESIAN_POINT('Ctrl Pts',(-21.2957664845097,19.4149927548523,-4.17674049236887));
#43801=CARTESIAN_POINT('Ctrl Pts',(-21.1817726734028,20.4667260333026,-4.22916299198858));
#43802=CARTESIAN_POINT('Ctrl Pts',(-19.7363287853609,22.0632999679849,-4.32362832418352));
#43803=CARTESIAN_POINT('Ctrl Pts',(-17.8395945320329,21.7565647566733,-4.40806309231925));
#43804=CARTESIAN_POINT('Ctrl Pts',(-17.1718943259273,21.2444859191099,-4.45010592489449));
#43805=CARTESIAN_POINT('Ctrl Pts',(-17.1744642439897,21.2411350264762,-3.6500459524789));
#43806=CARTESIAN_POINT('Ctrl Pts',(-17.1077769031899,21.189906270214,-3.65422167346473));
#43807=CARTESIAN_POINT('Ctrl Pts',(-17.0436659910486,21.1354262971526,-3.65839739445057));
#43808=CARTESIAN_POINT('Ctrl Pts',(-16.9824502029285,21.0779957976329,-3.66257311543641));
#43809=CARTESIAN_POINT('Ctrl Pts',(-16.9200837263783,21.0194857626965,-3.66682732849061));
#43810=CARTESIAN_POINT('Ctrl Pts',(-16.8607226752009,20.9579135054828,-3.6710815415448));
#43811=CARTESIAN_POINT('Ctrl Pts',(-16.8046620408575,20.8936333645247,-3.675335754599));
#43812=CARTESIAN_POINT('Ctrl Pts',(-16.748601406514,20.8293532235666,-3.6795899676532));
#43813=CARTESIAN_POINT('Ctrl Pts',(-16.6958414444482,20.7623656310848,-3.68384418070739));
#43814=CARTESIAN_POINT('Ctrl Pts',(-16.6466304638568,20.6930554711553,-3.68809839376159));
#43815=CARTESIAN_POINT('Ctrl Pts',(-16.5982243404927,20.6248788952851,-3.69228302815505));
#43816=CARTESIAN_POINT('Ctrl Pts',(-16.553071769447,20.5542014284547,-3.69646766254851));
#43817=CARTESIAN_POINT('Ctrl Pts',(-16.511440993796,20.4813666651567,-3.70065229694197));
#43818=CARTESIAN_POINT('Ctrl Pts',(-16.4698694744012,20.408635573129,-3.70483097502633));
#43819=CARTESIAN_POINT('Ctrl Pts',(-16.4318100196567,20.3337536798785,-3.70900965311069));
#43820=CARTESIAN_POINT('Ctrl Pts',(-16.3974886040357,20.2570948793148,-3.71318833119505));
#43821=CARTESIAN_POINT('Ctrl Pts',(-16.3625520017103,20.1790620248544,-3.71744190908038));
#43822=CARTESIAN_POINT('Ctrl Pts',(-16.3314890444374,20.0991883275089,-3.72169548696571));
#43823=CARTESIAN_POINT('Ctrl Pts',(-16.3044899883695,20.0178959681317,-3.72594906485105));
#43824=CARTESIAN_POINT('Ctrl Pts',(-16.2780143616845,19.9381796197598,-3.73012017882943));
#43825=CARTESIAN_POINT('Ctrl Pts',(-16.2554466207297,19.8570995822358,-3.73429129280781));
#43826=CARTESIAN_POINT('Ctrl Pts',(-16.2369175937363,19.7750739812545,-3.7384624067862));
#43827=CARTESIAN_POINT('Ctrl Pts',(-16.2183947843369,19.6930759047558,-3.74263212110701));
#43828=CARTESIAN_POINT('Ctrl Pts',(-16.2039080986716,19.6101333433017,-3.74680183542781));
#43829=CARTESIAN_POINT('Ctrl Pts',(-16.1935378668542,19.5266772878308,-3.75097154974862));
#43830=CARTESIAN_POINT('Ctrl Pts',(-16.1831680040541,19.4432242020846,-3.7551411156931));
#43831=CARTESIAN_POINT('Ctrl Pts',(-16.1769143597415,19.3592581152788,-3.75931068163757));
#43832=CARTESIAN_POINT('Ctrl Pts',(-16.174805548368,19.2752164989404,-3.76348024758204));
#43833=CARTESIAN_POINT('Ctrl Pts',(-16.1726225937887,19.1882200830672,-3.76779641032046));
#43834=CARTESIAN_POINT('Ctrl Pts',(-16.1748813730051,19.1011432548622,-3.77211257305887));
#43835=CARTESIAN_POINT('Ctrl Pts',(-16.1815548449752,19.0144707894735,-3.77642873579729));
#43836=CARTESIAN_POINT('Ctrl Pts',(-16.1880109292992,18.9306216705099,-3.78060429998941));
#43837=CARTESIAN_POINT('Ctrl Pts',(-16.1985983999137,18.8471514360449,-3.78477986418153));
#43838=CARTESIAN_POINT('Ctrl Pts',(-16.2132401674604,18.7644914707929,-3.78895542837364));
#43839=CARTESIAN_POINT('Ctrl Pts',(-16.2286214558733,18.6776565472299,-3.79334189038521));
#43840=CARTESIAN_POINT('Ctrl Pts',(-16.24847723842,18.5917164663179,-3.79772835239677));
#43841=CARTESIAN_POINT('Ctrl Pts',(-16.2726586407169,18.5071543400131,-3.80211481440834));
#43842=CARTESIAN_POINT('Ctrl Pts',(-16.2968400430138,18.4225922137084,-3.8065012764199));
#43843=CARTESIAN_POINT('Ctrl Pts',(-16.3253468050043,18.3394085662325,-3.81088773843146));
#43844=CARTESIAN_POINT('Ctrl Pts',(-16.3579723492966,18.2580610706385,-3.81527420044303));
#43845=CARTESIAN_POINT('Ctrl Pts',(-16.3890967439393,18.1804564938875,-3.81945883483596));
#43846=CARTESIAN_POINT('Ctrl Pts',(-16.4240850782656,18.1042339549061,-3.8236434692289));
#43847=CARTESIAN_POINT('Ctrl Pts',(-16.4627936385718,18.029804984853,-3.82782810362184));
#43848=CARTESIAN_POINT('Ctrl Pts',(-16.5014471020336,17.9554819552264,-3.83200678170567));
#43849=CARTESIAN_POINT('Ctrl Pts',(-16.5438100629349,17.8829478282646,-3.8361854597895));
#43850=CARTESIAN_POINT('Ctrl Pts',(-16.5896904513643,17.8125949944205,-3.84036413787333));
#43851=CARTESIAN_POINT('Ctrl Pts',(-16.6363932127842,17.740981136589,-3.84461771575879));
#43852=CARTESIAN_POINT('Ctrl Pts',(-16.6867405623486,17.6716279878895,-3.84887129364426));
#43853=CARTESIAN_POINT('Ctrl Pts',(-16.7404804948183,17.6049240421263,-3.85312487152972));
#43854=CARTESIAN_POINT('Ctrl Pts',(-16.7931785738305,17.5395132825159,-3.85729598550756));
#43855=CARTESIAN_POINT('Ctrl Pts',(-16.8491385640374,17.4766502972939,-3.86146709948541));
#43856=CARTESIAN_POINT('Ctrl Pts',(-16.9080797027397,17.4166714158068,-3.86563821346325));
#43857=CARTESIAN_POINT('Ctrl Pts',(-16.9670010631736,17.3567126608127,-3.8698079277835));
#43858=CARTESIAN_POINT('Ctrl Pts',(-17.0289012632126,17.299636415355,-3.87397764210376));
#43859=CARTESIAN_POINT('Ctrl Pts',(-17.0934613888502,17.2457435115673,-3.87814735642402));
#43860=CARTESIAN_POINT('Ctrl Pts',(-17.1580192171616,17.1918525255203,-3.88231692236795));
#43861=CARTESIAN_POINT('Ctrl Pts',(-17.2252364291767,17.1411449500709,-3.88648648831189));
#43862=CARTESIAN_POINT('Ctrl Pts',(-17.2947606690324,17.0938816404849,-3.89065605425582));
#43863=CARTESIAN_POINT('Ctrl Pts',(-17.3667292953982,17.0449566112366,-3.89497221699488));
#43864=CARTESIAN_POINT('Ctrl Pts',(-17.4411697620701,16.9997228515219,-3.89928837973393));
#43865=CARTESIAN_POINT('Ctrl Pts',(-17.5176598130624,16.9584200236971,-3.90360454247298));
#43866=CARTESIAN_POINT('Ctrl Pts',(-17.5916582086847,16.9184626311467,-3.90778010666456));
#43867=CARTESIAN_POINT('Ctrl Pts',(-17.6675742634443,16.8821841636526,-3.91195567085613));
#43868=CARTESIAN_POINT('Ctrl Pts',(-17.7450035240569,16.8497533016281,-3.9161312350477));
#43869=CARTESIAN_POINT('Ctrl Pts',(-17.8263435525593,16.815684433857,-3.92051769706049));
#43870=CARTESIAN_POINT('Ctrl Pts',(-17.9093531188143,16.7858622689057,-3.92490415907329));
#43871=CARTESIAN_POINT('Ctrl Pts',(-17.9935454192401,16.7604231263167,-3.92929062108608));
#43872=CARTESIAN_POINT('Ctrl Pts',(-18.077737719666,16.7349839837276,-3.93367708309888));
#43873=CARTESIAN_POINT('Ctrl Pts',(-18.1631121727116,16.7139279285856,-3.93806354511167));
#43874=CARTESIAN_POINT('Ctrl Pts',(-18.249172131343,16.6973289917387,-3.94245000712447));
#43875=CARTESIAN_POINT('Ctrl Pts',(-18.3312723437007,16.6814937965827,-3.94663464151747));
#43876=CARTESIAN_POINT('Ctrl Pts',(-18.4143019582716,16.6696556340513,-3.95081927591047));
#43877=CARTESIAN_POINT('Ctrl Pts',(-18.4978371529756,16.6619164176737,-3.95500391030348));
#43878=CARTESIAN_POINT('Ctrl Pts',(-18.5812534456693,16.6541882171128,-3.95918258838737));
#43879=CARTESIAN_POINT('Ctrl Pts',(-18.6651734349296,16.6505474159413,-3.96336126647126));
#43880=CARTESIAN_POINT('Ctrl Pts',(-18.7491632186827,16.651044907269,-3.96753994455515));
#43881=CARTESIAN_POINT('Ctrl Pts',(-18.8346584589486,16.6515513157714,-3.9717935224406));
#43882=CARTESIAN_POINT('Ctrl Pts',(-18.9202255470369,16.6563459251098,-3.97604710032605));
#43883=CARTESIAN_POINT('Ctrl Pts',(-19.0054014154824,16.6654271230872,-3.9803006782115));
#43884=CARTESIAN_POINT('Ctrl Pts',(-19.0889259835097,16.6743322643211,-3.98447179218939));
#43885=CARTESIAN_POINT('Ctrl Pts',(-19.172073887133,16.6873592186152,-3.98864290616729));
#43886=CARTESIAN_POINT('Ctrl Pts',(-19.2544103550733,16.7044539576675,-3.99281402014518));
#43887=CARTESIAN_POINT('Ctrl Pts',(-19.3367191942166,16.7215429604151,-3.9969837344655));
#43888=CARTESIAN_POINT('Ctrl Pts',(-19.4182166883869,16.7426969435999,-4.00115344878583));
#43889=CARTESIAN_POINT('Ctrl Pts',(-19.4984772632645,16.7678105857401,-4.00532316310615));
#43890=CARTESIAN_POINT('Ctrl Pts',(-19.5787349821264,16.7929233342292,-4.00949272905014));
#43891=CARTESIAN_POINT('Ctrl Pts',(-19.657755430421,16.8219953233348,-4.01366229499414));
#43892=CARTESIAN_POINT('Ctrl Pts',(-19.7351285466053,16.8548714735456,-4.01783186093814));
#43893=CARTESIAN_POINT('Ctrl Pts',(-19.8152220061065,16.8889035086417,-4.02214802367712));
#43894=CARTESIAN_POINT('Ctrl Pts',(-19.8935496523617,16.9270119844459,-4.02646418641609));
#43895=CARTESIAN_POINT('Ctrl Pts',(-19.9696814081002,16.9689715751857,-4.03078034915507));
#43896=CARTESIAN_POINT('Ctrl Pts',(-20.0433331799012,17.0095643366693,-4.0349559133467));
#43897=CARTESIAN_POINT('Ctrl Pts',(-20.114929550452,17.0537608783681,-4.03913147753832));
#43898=CARTESIAN_POINT('Ctrl Pts',(-20.1841097633275,17.1013124225843,-4.04330704172995));
#43899=CARTESIAN_POINT('Ctrl Pts',(-20.256784104298,17.1512656822579,-4.0476935037426));
#43900=CARTESIAN_POINT('Ctrl Pts',(-20.3267913293727,17.2049214186624,-4.05207996575526));
#43901=CARTESIAN_POINT('Ctrl Pts',(-20.3937533178436,17.2619440942068,-4.05646642776792));
#43902=CARTESIAN_POINT('Ctrl Pts',(-20.4607153063144,17.3189667697512,-4.06085288978058));
#43903=CARTESIAN_POINT('Ctrl Pts',(-20.524631688673,17.3793559306722,-4.06523935179324));
#43904=CARTESIAN_POINT('Ctrl Pts',(-20.5851713910718,17.4427340469043,-4.0696258138059));
#43905=CARTESIAN_POINT('Ctrl Pts',(-20.6421808499863,17.5024164036099,-4.07375648865202));
#43906=CARTESIAN_POINT('Ctrl Pts',(-20.6964202744402,17.5649836670307,-4.07788716349815));
#43907=CARTESIAN_POINT('Ctrl Pts',(-20.7475781317949,17.6301448177783,-4.08201783834428));
#43908=CARTESIAN_POINT('Ctrl Pts',(-20.7986699217384,17.6952218166719,-4.08614317866296));
#43909=CARTESIAN_POINT('Ctrl Pts',(-20.8466877493677,17.7628856907895,-4.09026851898165));
#43910=CARTESIAN_POINT('Ctrl Pts',(-20.8913569516644,17.8328088002366,-4.09439385930033));
#43911=CARTESIAN_POINT('Ctrl Pts',(-20.9359826817961,17.9026638603613,-4.09851518482883));
#43912=CARTESIAN_POINT('Ctrl Pts',(-20.977265999821,17.9747733973533,-4.10263651035733));
#43913=CARTESIAN_POINT('Ctrl Pts',(-21.0149735460515,18.0487781269426,-4.10675783588582));
#43914=CARTESIAN_POINT('Ctrl Pts',(-21.0526563884393,18.122734372836,-4.1108764613559));
#43915=CARTESIAN_POINT('Ctrl Pts',(-21.0867678956213,18.1985829265156,-4.11499508682597));
#43916=CARTESIAN_POINT('Ctrl Pts',(-21.117119754579,18.2759383788566,-4.11911371229604));
#43917=CARTESIAN_POINT('Ctrl Pts',(-21.1474714047475,18.3532932990728,-4.12323230943427));
#43918=CARTESIAN_POINT('Ctrl Pts',(-21.174063267692,18.4321546644581,-4.1273509065725));
#43919=CARTESIAN_POINT('Ctrl Pts',(-21.1967549321189,18.5121165016086,-4.13146950371073));
#43920=CARTESIAN_POINT('Ctrl Pts',(-21.2194452848828,18.5920737166658,-4.13558786277863));
#43921=CARTESIAN_POINT('Ctrl Pts',(-21.238235765403,18.6731308198826,-4.13970622184654));
#43922=CARTESIAN_POINT('Ctrl Pts',(-21.2530362470694,18.7548680169614,-4.14382458091445));
#43923=CARTESIAN_POINT('Ctrl Pts',(-21.2678499327185,18.8366781344066,-4.14794661410212));
#43924=CARTESIAN_POINT('Ctrl Pts',(-21.2786664327327,18.9191690901919,-4.1520686472898));
#43925=CARTESIAN_POINT('Ctrl Pts',(-21.2854471635996,19.001913005284,-4.15619068047748));
#43926=CARTESIAN_POINT('Ctrl Pts',(-21.2912151852698,19.0722990307271,-4.15969708372782));
#43927=CARTESIAN_POINT('Ctrl Pts',(-21.2940637843831,19.1428678239492,-4.16320348697816));
#43928=CARTESIAN_POINT('Ctrl Pts',(-21.2939989159607,19.2133559031925,-4.16670989022851));
#43929=CARTESIAN_POINT('Origin',(-18.734,19.211,1.76670989022852));
#43930=CARTESIAN_POINT('',(-17.1767158522682,21.2382341403344,-2.85017127940472));
#43931=CARTESIAN_POINT('',(-17.1744642439897,21.2411350264762,-2.91665630319145));
#43932=CARTESIAN_POINT('',(-17.1744642439897,21.2411350264762,1.76670989022852));
#43933=CARTESIAN_POINT('',(-21.2939999971965,19.2108801919503,-3.43329010980363));
#43934=CARTESIAN_POINT('Ctrl Pts',(-17.1744642439897,21.2411350264762,-2.91665630319145));
#43935=CARTESIAN_POINT('Ctrl Pts',(-17.1375641435127,21.2127886232351,-2.91898053472258));
#43936=CARTESIAN_POINT('Ctrl Pts',(-17.101470973183,21.1834618385403,-2.92130476625372));
#43937=CARTESIAN_POINT('Ctrl Pts',(-17.0662376770537,21.1532072068038,-2.92362899778485));
#43938=CARTESIAN_POINT('Ctrl Pts',(-17.002802317601,21.0987356230989,-2.92781363217408));
#43939=CARTESIAN_POINT('Ctrl Pts',(-16.9419203976439,21.0410515629429,-2.9319982665633));
#43940=CARTESIAN_POINT('Ctrl Pts',(-16.883935185605,20.9804236865537,-2.93618290095253));
#43941=CARTESIAN_POINT('Ctrl Pts',(-16.8260325083393,20.9198821064435,-2.94036157903258));
#43942=CARTESIAN_POINT('Ctrl Pts',(-16.7710186644539,20.8564053626863,-2.94454025711262));
#43943=CARTESIAN_POINT('Ctrl Pts',(-16.7192032202845,20.7903017243225,-2.94871893519267));
#43944=CARTESIAN_POINT('Ctrl Pts',(-16.6664590214564,20.7230132256709,-2.95297251307907));
#43945=CARTESIAN_POINT('Ctrl Pts',(-16.6170293785849,20.653003046041,-2.95722609096547));
#43946=CARTESIAN_POINT('Ctrl Pts',(-16.5712008555424,20.5806349370301,-2.96147966885187));
#43947=CARTESIAN_POINT('Ctrl Pts',(-16.5262608079,20.5096698251123,-2.96565078282577));
#43948=CARTESIAN_POINT('Ctrl Pts',(-16.4847837540961,20.4364378006271,-2.96982189679966));
#43949=CARTESIAN_POINT('Ctrl Pts',(-16.4469976092755,20.3613130290579,-2.97399301077356));
#43950=CARTESIAN_POINT('Ctrl Pts',(-16.4092241439612,20.2862134663323,-2.97816272508982));
#43951=CARTESIAN_POINT('Ctrl Pts',(-16.3751393344489,20.2092228285331,-2.98233243940609));
#43952=CARTESIAN_POINT('Ctrl Pts',(-16.3449251982357,20.1307399586702,-2.98650215372236));
#43953=CARTESIAN_POINT('Ctrl Pts',(-16.3147121371714,20.0522598815654,-2.99067171966225));
#43954=CARTESIAN_POINT('Ctrl Pts',(-16.2883696400355,19.9722881075971,-2.99484128560214));
#43955=CARTESIAN_POINT('Ctrl Pts',(-16.2660311035615,19.8912422555325,-2.99901085154203));
#43956=CARTESIAN_POINT('Ctrl Pts',(-16.2429071716539,19.8073469311139,-3.00332701428572));
#43957=CARTESIAN_POINT('Ctrl Pts',(-16.2240741377499,19.7223011025939,-3.00764317702941));
#43958=CARTESIAN_POINT('Ctrl Pts',(-16.2096228114109,19.6365817309648,-3.01195933977309));
#43959=CARTESIAN_POINT('Ctrl Pts',(-16.1956422355369,19.5536546590259,-3.01613490396055));
#43960=CARTESIAN_POINT('Ctrl Pts',(-16.1857622912647,19.4700977247645,-3.02031046814801));
#43961=CARTESIAN_POINT('Ctrl Pts',(-16.1800123293527,19.3863481627554,-3.02448603233547));
#43962=CARTESIAN_POINT('Ctrl Pts',(-16.173971950515,19.29836860919,-3.02887249435727));
#43963=CARTESIAN_POINT('Ctrl Pts',(-16.1724897391971,19.2101770410221,-3.03325895637908));
#43964=CARTESIAN_POINT('Ctrl Pts',(-16.175537874784,19.1222782223174,-3.03764541840088));
#43965=CARTESIAN_POINT('Ctrl Pts',(-16.1785860103709,19.0343794036126,-3.04203188042268));
#43966=CARTESIAN_POINT('Ctrl Pts',(-16.1861643670755,18.9467739058737,-3.04641834244449));
#43967=CARTESIAN_POINT('Ctrl Pts',(-16.1981829862585,18.8599557395154,-3.05080480446629));
#43968=CARTESIAN_POINT('Ctrl Pts',(-16.2096486109408,18.777132205804,-3.05498943886225));
#43969=CARTESIAN_POINT('Ctrl Pts',(-16.2251975483162,18.6947168580516,-3.0591740732582));
#43970=CARTESIAN_POINT('Ctrl Pts',(-16.244789702343,18.6131437513597,-3.06335870765416));
#43971=CARTESIAN_POINT('Ctrl Pts',(-16.2643539693637,18.5316867538876,-3.06753738574105));
#43972=CARTESIAN_POINT('Ctrl Pts',(-16.2879499152422,18.4510700597166,-3.07171606382794));
#43973=CARTESIAN_POINT('Ctrl Pts',(-16.3154858968848,18.3717208253311,-3.07589474191484));
#43974=CARTESIAN_POINT('Ctrl Pts',(-16.343515441184,18.2909493130174,-3.08014831979954));
#43975=CARTESIAN_POINT('Ctrl Pts',(-16.3756275947392,18.2114916234351,-3.08440189768424));
#43976=CARTESIAN_POINT('Ctrl Pts',(-16.4116716116104,18.1337856032898,-3.08865547556895));
#43977=CARTESIAN_POINT('Ctrl Pts',(-16.4470168449122,18.0575860659074,-3.09282658954992));
#43978=CARTESIAN_POINT('Ctrl Pts',(-16.4861426458307,17.9830713215449,-3.0969977035309));
#43979=CARTESIAN_POINT('Ctrl Pts',(-16.528857766551,17.9106355394507,-3.10116881751188));
#43980=CARTESIAN_POINT('Ctrl Pts',(-16.5715585538004,17.8382240638824,-3.1053385318353));
#43981=CARTESIAN_POINT('Ctrl Pts',(-16.6178460353512,17.7678905610413,-3.10950824615873));
#43982=CARTESIAN_POINT('Ctrl Pts',(-16.6674833699683,17.7000039649946,-3.11367796048215));
#43983=CARTESIAN_POINT('Ctrl Pts',(-16.7171189382761,17.632119784644,-3.11784752642926));
#43984=CARTESIAN_POINT('Ctrl Pts',(-16.7701038504313,17.5666827088182,-3.12201709237638));
#43985=CARTESIAN_POINT('Ctrl Pts',(-16.8261591602606,17.504030952178,-3.12618665832349));
#43986=CARTESIAN_POINT('Ctrl Pts',(-16.8841853055411,17.4391764371649,-3.13050282105884));
#43987=CARTESIAN_POINT('Ctrl Pts',(-16.9455014243886,17.3773071422649,-3.13481898379419));
#43988=CARTESIAN_POINT('Ctrl Pts',(-17.009755621585,17.3187575938839,-3.13913514652954));
#43989=CARTESIAN_POINT('Ctrl Pts',(-17.0719167451634,17.2621152907944,-3.14331071072431));
#43990=CARTESIAN_POINT('Ctrl Pts',(-17.1368270773952,17.2085800374251,-3.14748627491907));
#43991=CARTESIAN_POINT('Ctrl Pts',(-17.2041348602048,17.1584131799021,-3.15166183911384));
#43992=CARTESIAN_POINT('Ctrl Pts',(-17.2748421989517,17.1057125137878,-3.15604830111948));
#43993=CARTESIAN_POINT('Ctrl Pts',(-17.3481950580309,17.0567297857013,-3.16043476312513));
#43994=CARTESIAN_POINT('Ctrl Pts',(-17.4237539519783,17.0117148221198,-3.16482122513078));
#43995=CARTESIAN_POINT('Ctrl Pts',(-17.4993128459257,16.9666998585384,-3.16920768713642));
#43996=CARTESIAN_POINT('Ctrl Pts',(-17.5770772261119,16.9256528630385,-3.17359414914207));
#43997=CARTESIAN_POINT('Ctrl Pts',(-17.6565830150582,16.8887655931067,-3.17798061114772));
#43998=CARTESIAN_POINT('Ctrl Pts',(-17.7324306249075,16.8535755610943,-3.18216524554016));
#43999=CARTESIAN_POINT('Ctrl Pts',(-17.8101452346757,16.8220398921685,-3.18634987993261));
#44000=CARTESIAN_POINT('Ctrl Pts',(-17.8893401694872,16.7943598176977,-3.19053451432505));
#44001=CARTESIAN_POINT('Ctrl Pts',(-17.9684223801113,16.7667191423868,-3.19471319240839));
#44002=CARTESIAN_POINT('Ctrl Pts',(-18.0489802999387,16.7429233111999,-3.19889187049172));
#44003=CARTESIAN_POINT('Ctrl Pts',(-18.1306051532975,16.7231264785016,-3.20307054857506));
#44004=CARTESIAN_POINT('Ctrl Pts',(-18.213693073505,16.7029748018013,-3.20732412646065));
#44005=CARTESIAN_POINT('Ctrl Pts',(-18.2978861156729,16.6869671007255,-3.21157770434623));
#44006=CARTESIAN_POINT('Ctrl Pts',(-18.3827345240937,16.6752136199127,-3.21583128223182));
#44007=CARTESIAN_POINT('Ctrl Pts',(-18.4659379805341,16.6636880032625,-3.22000239620916));
#44008=CARTESIAN_POINT('Ctrl Pts',(-18.5497711422168,16.6562531921902,-3.22417351018651));
#44009=CARTESIAN_POINT('Ctrl Pts',(-18.6337990563682,16.6529617338876,-3.22834462416385));
#44010=CARTESIAN_POINT('Ctrl Pts',(-18.7177987741416,16.6496713800656,-3.23251433848362));
#44011=CARTESIAN_POINT('Ctrl Pts',(-18.8019926552976,16.6505216357632,-3.23668405280339));
#44012=CARTESIAN_POINT('Ctrl Pts',(-18.885942287003,16.6555130519957,-3.24085376712315));
#44013=CARTESIAN_POINT('Ctrl Pts',(-18.9698889314202,16.6605042906123,-3.24502333306659));
#44014=CARTESIAN_POINT('Ctrl Pts',(-19.0535908844962,16.669636368619,-3.24919289901003));
#44015=CARTESIAN_POINT('Ctrl Pts',(-19.1366127729526,16.6828578056099,-3.25336246495347));
#44016=CARTESIAN_POINT('Ctrl Pts',(-19.2225536086153,16.6965440920193,-3.25767862769311));
#44017=CARTESIAN_POINT('Ctrl Pts',(-19.3077651468771,16.7146125685867,-3.26199479043275));
#44018=CARTESIAN_POINT('Ctrl Pts',(-19.3917756297612,16.7369484199208,-3.26631095317239));
#44019=CARTESIAN_POINT('Ctrl Pts',(-19.4730494799765,16.7585566832404,-3.27048651736348));
#44020=CARTESIAN_POINT('Ctrl Pts',(-19.5531988875823,16.7841583830433,-3.27466208155456));
#44021=CARTESIAN_POINT('Ctrl Pts',(-19.6318137018712,16.8135992081564,-3.27883764574565));
#44022=CARTESIAN_POINT('Ctrl Pts',(-19.7143991635786,16.8445270193712,-3.28322410775957));
#44023=CARTESIAN_POINT('Ctrl Pts',(-19.7952903977548,16.8796917438777,-3.28761056977348));
#44024=CARTESIAN_POINT('Ctrl Pts',(-19.8740394547192,16.9188590702831,-3.2919970317874));
#44025=CARTESIAN_POINT('Ctrl Pts',(-19.9527885116835,16.9580263966884,-3.29638349380132));
#44026=CARTESIAN_POINT('Ctrl Pts',(-20.0293949232977,17.0011959738741,-3.30076995581524));
#44027=CARTESIAN_POINT('Ctrl Pts',(-20.1034462555219,17.0480813808104,-3.30515641782916));
#44028=CARTESIAN_POINT('Ctrl Pts',(-20.1740903761505,17.092809520654,-3.30934105222176));
#44029=CARTESIAN_POINT('Ctrl Pts',(-20.2426723273843,17.1410855493988,-3.31352568661436));
#44030=CARTESIAN_POINT('Ctrl Pts',(-20.3088136057117,17.19269325739,-3.31771032100697));
#44031=CARTESIAN_POINT('Ctrl Pts',(-20.374860740116,17.2442275081965,-3.32188899909046));
#44032=CARTESIAN_POINT('Ctrl Pts',(-20.4384737424745,17.2990837381083,-3.32606767717394));
#44033=CARTESIAN_POINT('Ctrl Pts',(-20.4993017308437,17.3570016723092,-3.33024635525743));
#44034=CARTESIAN_POINT('Ctrl Pts',(-20.5612200171964,17.4159577438638,-3.33449993314298));
#44035=CARTESIAN_POINT('Ctrl Pts',(-20.6202520574043,17.4780861035065,-3.33875351102853));
#44036=CARTESIAN_POINT('Ctrl Pts',(-20.6760617089389,17.5430682511945,-3.34300708891408));
#44037=CARTESIAN_POINT('Ctrl Pts',(-20.7307893814672,17.6067905931385,-3.34717820289156));
#44038=CARTESIAN_POINT('Ctrl Pts',(-20.7824181813928,17.6732566930095,-3.35134931686903));
#44039=CARTESIAN_POINT('Ctrl Pts',(-20.8306684931563,17.742129267156,-3.35552043084651));
#44040=CARTESIAN_POINT('Ctrl Pts',(-20.8789026140616,17.810978730445,-3.3596901451664));
#44041=CARTESIAN_POINT('Ctrl Pts',(-20.923760234583,17.8822326878121,-3.36385985948629));
#44042=CARTESIAN_POINT('Ctrl Pts',(-20.9650035868519,17.955522801699,-3.36802957380618));
#44043=CARTESIAN_POINT('Ctrl Pts',(-21.0062454715054,18.028810307609,-3.37219913974974));
#44044=CARTESIAN_POINT('Ctrl Pts',(-21.0438731187515,18.1041334246492,-3.37636870569329));
#44045=CARTESIAN_POINT('Ctrl Pts',(-21.0776941561666,18.1810982074244,-3.38053827163685));
#44046=CARTESIAN_POINT('Ctrl Pts',(-21.1127042995431,18.2607689770352,-3.38485443437633));
#44047=CARTESIAN_POINT('Ctrl Pts',(-21.1436349596428,18.3421985193634,-3.3891705971158));
#44048=CARTESIAN_POINT('Ctrl Pts',(-21.1703273243944,18.4249280132143,-3.39348675985528));
#44049=CARTESIAN_POINT('Ctrl Pts',(-21.1961501881654,18.5049626024847,-3.39766232404647));
#44050=CARTESIAN_POINT('Ctrl Pts',(-21.2180065643708,18.5862132848946,-3.40183788823765));
#44051=CARTESIAN_POINT('Ctrl Pts',(-21.2358041974883,18.6682516628954,-3.40601345242883));
#44052=CARTESIAN_POINT('Ctrl Pts',(-21.2545007467516,18.7544336043729,-3.41039991444246));
#44053=CARTESIAN_POINT('Ctrl Pts',(-21.2687176692139,18.8414843294195,-3.41478637645609));
#44054=CARTESIAN_POINT('Ctrl Pts',(-21.2784095170101,18.9289003549305,-3.41917283846971));
#44055=CARTESIAN_POINT('Ctrl Pts',(-21.2881013648063,19.0163163804415,-3.42355930048334));
#44056=CARTESIAN_POINT('Ctrl Pts',(-21.293268179777,19.1040971227328,-3.42794576249697));
#44057=CARTESIAN_POINT('Ctrl Pts',(-21.2939275539577,19.1917407557754,-3.43233222451059));
#44058=CARTESIAN_POINT('Ctrl Pts',(-21.2939755504833,19.1981204260763,-3.43265151959756));
#44059=CARTESIAN_POINT('Ctrl Pts',(-21.2939996986147,19.2045002760229,-3.43297081468453));
#44060=CARTESIAN_POINT('Ctrl Pts',(-21.2939999971965,19.2108801913083,-3.4332901097715));
#44061=CARTESIAN_POINT('Ctrl Pts',(-21.2939999971965,19.2108801919503,-3.43329010980363));
#44062=CARTESIAN_POINT('Ctrl Pts',(-21.294003905102,19.2943824116244,-3.43746913841141));
#44063=CARTESIAN_POINT('Ctrl Pts',(-21.2899179933662,19.3780422026729,-3.44164816701919));
#44064=CARTESIAN_POINT('Ctrl Pts',(-21.2817219740999,19.4614251239161,-3.44582719562696));
#44065=CARTESIAN_POINT('Ctrl Pts',(-21.2735376207105,19.5446893613373,-3.45000027597723));
#44066=CARTESIAN_POINT('Ctrl Pts',(-21.2612548239782,19.6276770564323,-3.45417335632749));
#44067=CARTESIAN_POINT('Ctrl Pts',(-21.2449053023278,19.7099534675119,-3.45834643667776));
#44068=CARTESIAN_POINT('Ctrl Pts',(-21.228391285294,19.7930576758855,-3.46256150311585));
#44069=CARTESIAN_POINT('Ctrl Pts',(-21.2077282378307,19.875435728573,-3.46677656955395));
#44070=CARTESIAN_POINT('Ctrl Pts',(-21.1830026840864,19.9566445891559,-3.47099163599204));
#44071=CARTESIAN_POINT('Ctrl Pts',(-21.1585674190593,20.0369000225192,-3.47515721572332));
#44072=CARTESIAN_POINT('Ctrl Pts',(-21.1301646741428,20.1160131199896,-3.47932279545459));
#44073=CARTESIAN_POINT('Ctrl Pts',(-21.0979289771719,20.1935679573886,-3.48348837518587));
#44074=CARTESIAN_POINT('Ctrl Pts',(-21.0657039544922,20.2710971138504,-3.48765257555778));
#44075=CARTESIAN_POINT('Ctrl Pts',(-21.0296486772609,20.347068609211,-3.49181677592968));
#44076=CARTESIAN_POINT('Ctrl Pts',(-20.9899463178963,20.4210852080619,-3.49598097630159));
#44077=CARTESIAN_POINT('Ctrl Pts',(-20.9502451090693,20.4950996619801,-3.50014505599882));
#44078=CARTESIAN_POINT('Ctrl Pts',(-20.9068972472216,20.5671589258642,-3.50430913569605));
#44079=CARTESIAN_POINT('Ctrl Pts',(-20.8601318431733,20.6368903833901,-3.50847321539329));
#44080=CARTESIAN_POINT('Ctrl Pts',(-20.8123689128483,20.7081092430375,-3.51272611670985));
#44081=CARTESIAN_POINT('Ctrl Pts',(-20.7610412266545,20.7768994173757,-3.51697901802641));
#44082=CARTESIAN_POINT('Ctrl Pts',(-20.7064383509255,20.8428967344162,-3.52123191934297));
#44083=CARTESIAN_POINT('Ctrl Pts',(-20.6528987388227,20.9076089076671,-3.52540200532764));
#44084=CARTESIAN_POINT('Ctrl Pts',(-20.5962107113947,20.969635714652,-3.5295720913123));
#44085=CARTESIAN_POINT('Ctrl Pts',(-20.5366855500212,21.0286701592271,-3.53374217729697));
#44086=CARTESIAN_POINT('Ctrl Pts',(-20.4753871892413,21.0894631852098,-3.53803648627948));
#44087=CARTESIAN_POINT('Ctrl Pts',(-20.411080380652,21.1470823903906,-3.54233079526199));
#44088=CARTESIAN_POINT('Ctrl Pts',(-20.3441412203941,21.2012374859267,-3.54662510424449));
#44089=CARTESIAN_POINT('Ctrl Pts',(-20.2772020601362,21.2553925814628,-3.550919413227));
#44090=CARTESIAN_POINT('Ctrl Pts',(-20.2076310154016,21.306083314333,-3.55521372220951));
#44091=CARTESIAN_POINT('Ctrl Pts',(-20.1358342086543,21.353069291934,-3.55950803119202));
#44092=CARTESIAN_POINT('Ctrl Pts',(-20.0658710578792,21.3988552702266,-3.56369266558496));
#44093=CARTESIAN_POINT('Ctrl Pts',(-19.9935321931099,21.4412951999105,-3.56787729997789));
#44094=CARTESIAN_POINT('Ctrl Pts',(-19.9191711337672,21.4801340603157,-3.57206193437083));
#44095=CARTESIAN_POINT('Ctrl Pts',(-19.8449159181885,21.5189176384104,-3.57624061245465));
#44096=CARTESIAN_POINT('Ctrl Pts',(-19.7686446296092,21.5541101172785,-3.58041929053848));
#44097=CARTESIAN_POINT('Ctrl Pts',(-19.690739462204,21.5854998634368,-3.58459796862231));
#44098=CARTESIAN_POINT('Ctrl Pts',(-19.6114379006597,21.6174522482367,-3.58885154650778));
#44099=CARTESIAN_POINT('Ctrl Pts',(-19.5304437130248,21.645463967428,-3.59310512439324));
#44100=CARTESIAN_POINT('Ctrl Pts',(-19.4481859912097,21.6693609112496,-3.5973587022787));
#44101=CARTESIAN_POINT('Ctrl Pts',(-19.3675229958474,21.6927945661833,-3.60152981625654));
#44102=CARTESIAN_POINT('Ctrl Pts',(-19.2856454833722,21.7122714336375,-3.60570093023438));
#44103=CARTESIAN_POINT('Ctrl Pts',(-19.2029762398825,21.7276766352524,-3.60987204421221));
#44104=CARTESIAN_POINT('Ctrl Pts',(-19.1203347368559,21.7430766675032,-3.61404175853247));
#44105=CARTESIAN_POINT('Ctrl Pts',(-19.0369024823169,21.754407663177,-3.61821147285273));
#44106=CARTESIAN_POINT('Ctrl Pts',(-18.9531132034118,21.7616056935737,-3.62238118717299));
#44107=CARTESIAN_POINT('Ctrl Pts',(-18.8693269060889,21.7688034678336,-3.62655075311692));
#44108=CARTESIAN_POINT('Ctrl Pts',(-18.7851840680773,21.7718685307012,-3.63072031906085));
#44109=CARTESIAN_POINT('Ctrl Pts',(-18.7011229313379,21.7707888776921,-3.63488988500478));
#44110=CARTESIAN_POINT('Ctrl Pts',(-18.6141063087263,21.769671265415,-3.63920604774384));
#44111=CARTESIAN_POINT('Ctrl Pts',(-18.5271777668963,21.7641120647909,-3.6435222104829));
#44112=CARTESIAN_POINT('Ctrl Pts',(-18.4408207068909,21.7541566806023,-3.64783837322195));
#44113=CARTESIAN_POINT('Ctrl Pts',(-18.3572767190368,21.744525592007,-3.65201393741352));
#44114=CARTESIAN_POINT('Ctrl Pts',(-18.2742680097319,21.7307804563761,-3.65618950160509));
#44115=CARTESIAN_POINT('Ctrl Pts',(-18.1922227301014,21.7130146661883,-3.66036506579665));
#44116=CARTESIAN_POINT('Ctrl Pts',(-18.1060335384334,21.6943515681706,-3.66475152780945));
#44117=CARTESIAN_POINT('Ctrl Pts',(-18.0209082233735,21.6712511277376,-3.66913798982225));
#44118=CARTESIAN_POINT('Ctrl Pts',(-17.937323903919,21.6438804323133,-3.67352445183506));
#44119=CARTESIAN_POINT('Ctrl Pts',(-17.8537395844645,21.616509736889,-3.67791091384786));
#44120=CARTESIAN_POINT('Ctrl Pts',(-17.7716967745983,21.584869066222,-3.68229737586066));
#44121=CARTESIAN_POINT('Ctrl Pts',(-17.6916449845522,21.5491822045706,-3.68668383787346));
#44122=CARTESIAN_POINT('Ctrl Pts',(-17.6152736995615,21.5151361016662,-3.69086862550016));
#44123=CARTESIAN_POINT('Ctrl Pts',(-17.5404300949785,21.4772809673625,-3.69505341312687));
#44124=CARTESIAN_POINT('Ctrl Pts',(-17.4675200004595,21.4357760360908,-3.69923820075358));
#44125=CARTESIAN_POINT('Ctrl Pts',(-17.3947226531712,21.39433528751,-3.70341651707862));
#44126=CARTESIAN_POINT('Ctrl Pts',(-17.3238532702767,21.3492561841251,-3.70759483340367));
#44127=CARTESIAN_POINT('Ctrl Pts',(-17.2552965767404,21.3007454835554,-3.71177314972872));
#44128=CARTESIAN_POINT('Ctrl Pts',(-17.227977727748,21.2814146722952,-3.71343814824073));
#44129=CARTESIAN_POINT('Ctrl Pts',(-17.2010258627729,21.2615394792291,-3.71510314675274));
#44130=CARTESIAN_POINT('Ctrl Pts',(-17.1744642439897,21.2411350264762,-3.71676814526475));
#44131=CARTESIAN_POINT('',(-21.2936055426903,19.2106176052578,-3.36670986511441));
#44132=CARTESIAN_POINT('Ctrl Pts',(-21.2939999715072,19.2106180532905,-3.36670989022851));
#44133=CARTESIAN_POINT('Ctrl Pts',(-21.2940130064034,19.2979845189442,-3.37103154303559));
#44134=CARTESIAN_POINT('Ctrl Pts',(-21.2895493128086,19.3852864628676,-3.37535319584268));
#44135=CARTESIAN_POINT('Ctrl Pts',(-21.2806546261691,19.4720559614555,-3.37967484864976));
#44136=CARTESIAN_POINT('Ctrl Pts',(-21.2713805337796,19.5625266412119,-3.38418084296218));
#44137=CARTESIAN_POINT('Ctrl Pts',(-21.2572890869444,19.6524179424097,-3.38868683727459));
#44138=CARTESIAN_POINT('Ctrl Pts',(-21.2384911684206,19.7412112666692,-3.393192831587));
#44139=CARTESIAN_POINT('Ctrl Pts',(-21.2204017935413,19.8266577339088,-3.3975289829656));
#44140=CARTESIAN_POINT('Ctrl Pts',(-21.1979545494935,19.911087135192,-3.40186513434419));
#44141=CARTESIAN_POINT('Ctrl Pts',(-21.1712990035409,19.9940540002698,-3.40620128572279));
#44142=CARTESIAN_POINT('Ctrl Pts',(-21.1446099328528,20.0771252129461,-3.41054289068797));
#44143=CARTESIAN_POINT('Ctrl Pts',(-21.1137021554183,20.1587298407179,-3.41488449565315));
#44144=CARTESIAN_POINT('Ctrl Pts',(-21.0787731611217,20.2384428562617,-3.41922610061834));
#44145=CARTESIAN_POINT('Ctrl Pts',(-21.0437703953367,20.3183242290092,-3.42357687523375));
#44146=CARTESIAN_POINT('Ctrl Pts',(-21.0047296348366,20.3963056454717,-3.42792764984916));
#44147=CARTESIAN_POINT('Ctrl Pts',(-20.9618940508659,20.4719869539834,-3.43227842446457));
#44148=CARTESIAN_POINT('Ctrl Pts',(-20.9570751477604,20.4805009243513,-3.43276787644263));
#44149=CARTESIAN_POINT('Ctrl Pts',(-20.9522082623986,20.4889858169837,-3.43325732842068));
#44150=CARTESIAN_POINT('Ctrl Pts',(-20.9472937739975,20.4974410868688,-3.43374678039873));
#44151=CARTESIAN_POINT('Ctrl Pts',(-20.9052767057113,20.5697305345463,-3.43793141479118));
#44152=CARTESIAN_POINT('Ctrl Pts',(-20.8596361007269,20.6400938357955,-3.44211604918362));
#44153=CARTESIAN_POINT('Ctrl Pts',(-20.8105736599315,20.7081445604478,-3.44630068357607));
#44154=CARTESIAN_POINT('Ctrl Pts',(-20.7615810534479,20.7760984233165,-3.45047936165941));
#44155=CARTESIAN_POINT('Ctrl Pts',(-20.7091765523538,20.8417458779045,-3.45465803974274));
#44156=CARTESIAN_POINT('Ctrl Pts',(-20.6536069384425,20.9047264247462,-3.45883671782608));
#44157=CARTESIAN_POINT('Ctrl Pts',(-20.5970412791288,20.9688358526382,-3.46309029571167));
#44158=CARTESIAN_POINT('Ctrl Pts',(-20.5371961639062,21.0301814068962,-3.46734387359725));
#44159=CARTESIAN_POINT('Ctrl Pts',(-20.4743771168498,21.0884151089052,-3.47159745148284));
#44160=CARTESIAN_POINT('Ctrl Pts',(-20.412775939613,21.1455198369568,-3.47576856546018));
#44161=CARTESIAN_POINT('Ctrl Pts',(-20.3483154653815,21.1996319675306,-3.47993967943753));
#44162=CARTESIAN_POINT('Ctrl Pts',(-20.2813221318913,21.250459296029,-3.48411079341487));
#44163=CARTESIAN_POINT('Ctrl Pts',(-20.2143512786613,21.3012695689265,-3.48828050773464));
#44164=CARTESIAN_POINT('Ctrl Pts',(-20.1448496203246,21.3487969510057,-3.4924502220544));
#44165=CARTESIAN_POINT('Ctrl Pts',(-20.0731762130974,21.3927898776633,-3.49661993637416));
#44166=CARTESIAN_POINT('Ctrl Pts',(-20.0015053563176,21.4367812388638,-3.50078950231759));
#44167=CARTESIAN_POINT('Ctrl Pts',(-19.9276632968144,21.4772381547836,-3.50495906826103));
#44168=CARTESIAN_POINT('Ctrl Pts',(-19.8520364016656,21.5139534525367,-3.50912863420446));
#44169=CARTESIAN_POINT('Ctrl Pts',(-19.7737505581546,21.5519596148775,-3.5134447969441));
#44170=CARTESIAN_POINT('Ctrl Pts',(-19.6935525085944,21.585955922694,-3.51776095968374));
#44171=CARTESIAN_POINT('Ctrl Pts',(-19.6118947218442,21.6157662791544,-3.52207712242338));
#44172=CARTESIAN_POINT('Ctrl Pts',(-19.5328969289329,21.6446055663797,-3.52625268661447));
#44173=CARTESIAN_POINT('Ctrl Pts',(-19.4525335041393,21.6695273345314,-3.53042825080555));
#44174=CARTESIAN_POINT('Ctrl Pts',(-19.3712290384541,21.690423149152,-3.53460381499664));
#44175=CARTESIAN_POINT('Ctrl Pts',(-19.2858180774511,21.712374361704,-3.53899027701056));
#44176=CARTESIAN_POINT('Ctrl Pts',(-19.1993690855429,21.7298821146793,-3.54337673902448));
#44177=CARTESIAN_POINT('Ctrl Pts',(-19.1123834602667,21.7428819002861,-3.5477632010384));
#44178=CARTESIAN_POINT('Ctrl Pts',(-19.0253978349904,21.755881685893,-3.55214966305232));
#44179=CARTESIAN_POINT('Ctrl Pts',(-18.9378761611969,21.7643735238079,-3.55653612506624));
#44180=CARTESIAN_POINT('Ctrl Pts',(-18.8503205710795,21.7683559636358,-3.56092258708016));
#44181=CARTESIAN_POINT('Ctrl Pts',(-18.7668123251272,21.7721543112249,-3.56510628052826));
#44182=CARTESIAN_POINT('Ctrl Pts',(-18.6829624657632,21.7718650921498,-3.56928997397637));
#44183=CARTESIAN_POINT('Ctrl Pts',(-18.599204802892,21.7674487585001,-3.57347366742447));
#44184=CARTESIAN_POINT('Ctrl Pts',(-18.5155577245013,21.7630382556955,-3.57765183718017));
#44185=CARTESIAN_POINT('Ctrl Pts',(-18.4320030559613,21.7545114802022,-3.58183000693587));
#44186=CARTESIAN_POINT('Ctrl Pts',(-18.3489773389754,21.7418807855167,-3.58600817669157));
#44187=CARTESIAN_POINT('Ctrl Pts',(-18.2660363238681,21.7292629765201,-3.59018208392669));
#44188=CARTESIAN_POINT('Ctrl Pts',(-18.183623640842,21.7125496319968,-3.59435599116181));
#44189=CARTESIAN_POINT('Ctrl Pts',(-18.1021720695873,21.6918050036934,-3.59852989839693));
#44190=CARTESIAN_POINT('Ctrl Pts',(-18.0183963786608,21.6704684531229,-3.60282290290376));
#44191=CARTESIAN_POINT('Ctrl Pts',(-17.9356379804305,21.6448670989516,-3.60711590741059));
#44192=CARTESIAN_POINT('Ctrl Pts',(-17.8543574465608,21.6151274879213,-3.61140891191742));
#44193=CARTESIAN_POINT('Ctrl Pts',(-17.775411049397,21.5862419106236,-3.61557863402291));
#44194=CARTESIAN_POINT('Ctrl Pts',(-17.6978592336747,21.5534527314071,-3.61974835612839));
#44195=CARTESIAN_POINT('Ctrl Pts',(-17.6221076884281,21.5169261669592,-3.62391807823388));
#44196=CARTESIAN_POINT('Ctrl Pts',(-17.5429966270672,21.4787796806806,-3.62827272394138));
#44197=CARTESIAN_POINT('Ctrl Pts',(-17.4658497272794,21.4365568045564,-3.63262736964889));
#44198=CARTESIAN_POINT('Ctrl Pts',(-17.3911027171311,21.3905015227485,-3.63698201535639));
#44199=CARTESIAN_POINT('Ctrl Pts',(-17.3163557069827,21.3444462409407,-3.64133666106389));
#44200=CARTESIAN_POINT('Ctrl Pts',(-17.244009058728,21.2945588745528,-3.64569130677139));
#44201=CARTESIAN_POINT('Ctrl Pts',(-17.1744642439897,21.2411350264762,-3.6500459524789));
#44202=CARTESIAN_POINT('Ctrl Pts',(-17.1767158522682,21.2382341403344,-2.85017127940472));
#44203=CARTESIAN_POINT('Ctrl Pts',(-16.7788810867994,20.9296544485643,-2.87512870416081));
#44204=CARTESIAN_POINT('Ctrl Pts',(-15.9356497699281,19.7924127402861,-2.94247806447738));
#44205=CARTESIAN_POINT('Ctrl Pts',(-16.3642904626609,17.3274479445074,-3.05221936035442));
#44206=CARTESIAN_POINT('Ctrl Pts',(-19.0350903727826,16.1989182890321,-3.17939516703585));
#44207=CARTESIAN_POINT('Ctrl Pts',(-21.0089154299348,17.5465283377359,-3.28422525530949));
#44208=CARTESIAN_POINT('Ctrl Pts',(-21.290373212379,18.8060182046973,-3.34666340802265));
#44209=CARTESIAN_POINT('Ctrl Pts',(-21.2898371856445,19.2106133247715,-3.36670962517532));
#44210=CARTESIAN_POINT('Origin',(-18.734,19.211,1.76670989022852));
#44211=CARTESIAN_POINT('',(-17.1744642439897,21.2411350264762,-2.05017636798559));
#44212=CARTESIAN_POINT('',(-17.1744642439897,21.2411350264762,-2.11663750951706));
#44213=CARTESIAN_POINT('',(-17.1744642439897,21.2411350264762,1.76670989022852));
#44214=CARTESIAN_POINT('',(-21.2939989850552,19.2132795868247,-2.63329010980608));
#44215=CARTESIAN_POINT('Ctrl Pts',(-17.1744642439897,21.2411350264762,-2.11663750951706));
#44216=CARTESIAN_POINT('Ctrl Pts',(-17.1077529033479,21.1898878337006,-2.1208121744548));
#44217=CARTESIAN_POINT('Ctrl Pts',(-17.0436084091249,21.135378288778,-2.12498683939254));
#44218=CARTESIAN_POINT('Ctrl Pts',(-16.9823526577971,21.0779042794298,-2.12916150433028));
#44219=CARTESIAN_POINT('Ctrl Pts',(-16.9210595534414,21.0203952231151,-2.13333871492899));
#44220=CARTESIAN_POINT('Ctrl Pts',(-16.8626590177325,20.9599184348882,-2.13751592552771));
#44221=CARTESIAN_POINT('Ctrl Pts',(-16.8074346248094,20.8968071820694,-2.14169313612642));
#44222=CARTESIAN_POINT('Ctrl Pts',(-16.7521184910976,20.8335910865205,-2.14587728606073));
#44223=CARTESIAN_POINT('Ctrl Pts',(-16.6999893181143,20.7677321503202,-2.15006143599504));
#44224=CARTESIAN_POINT('Ctrl Pts',(-16.6512888568846,20.6995947381148,-2.15424558592935));
#44225=CARTESIAN_POINT('Ctrl Pts',(-16.6267355331262,20.6652418819056,-2.15635510985165));
#44226=CARTESIAN_POINT('Ctrl Pts',(-16.6030530382591,20.6303102941139,-2.15846463377395));
#44227=CARTESIAN_POINT('Ctrl Pts',(-16.5802679097319,20.5948490103148,-2.16057415769624));
#44228=CARTESIAN_POINT('Ctrl Pts',(-16.5350693576789,20.5245049400697,-2.16475879184019));
#44229=CARTESIAN_POINT('Ctrl Pts',(-16.4932366287838,20.4518132565164,-2.16894342598413));
#44230=CARTESIAN_POINT('Ctrl Pts',(-16.455021774691,20.3771296019601,-2.17312806012807));
#44231=CARTESIAN_POINT('Ctrl Pts',(-16.4168613147564,20.3025522504267,-2.17730673795852));
#44232=CARTESIAN_POINT('Ctrl Pts',(-16.3823087086575,20.2259889657712,-2.18148541578897));
#44233=CARTESIAN_POINT('Ctrl Pts',(-16.3515723822767,20.1478237007618,-2.18566409361941));
#44234=CARTESIAN_POINT('Ctrl Pts',(-16.3202851269751,20.0682573735515,-2.18991767156768));
#44235=CARTESIAN_POINT('Ctrl Pts',(-16.2929525719374,19.9870314754769,-2.19417124951594));
#44236=CARTESIAN_POINT('Ctrl Pts',(-16.2697452279947,19.9045765413053,-2.1984248274642));
#44237=CARTESIAN_POINT('Ctrl Pts',(-16.2469878054675,19.823720163211,-2.20259594117975));
#44238=CARTESIAN_POINT('Ctrl Pts',(-16.2281972006316,19.7416824416901,-2.2067670548953));
#44239=CARTESIAN_POINT('Ctrl Pts',(-16.2134847477526,19.6588871098706,-2.21093816861086));
#44240=CARTESIAN_POINT('Ctrl Pts',(-16.1987772317893,19.5761195608808,-2.21510788266607));
#44241=CARTESIAN_POINT('Ctrl Pts',(-16.1881452304062,19.4925953590458,-2.21927759672128));
#44242=CARTESIAN_POINT('Ctrl Pts',(-16.1816490383842,19.4087487515486,-2.22344731077649));
#44243=CARTESIAN_POINT('Ctrl Pts',(-16.1751530775284,19.3249051277225,-2.22761687645295));
#44244=CARTESIAN_POINT('Ctrl Pts',(-16.1727926681034,19.2407395797693,-2.23178644212941));
#44245=CARTESIAN_POINT('Ctrl Pts',(-16.1745761446913,19.1566904347581,-2.23595600780587));
#44246=CARTESIAN_POINT('Ctrl Pts',(-16.1764223263664,19.0696862136873,-2.24027217085352));
#44247=CARTESIAN_POINT('Ctrl Pts',(-16.1827092038737,18.982807260651,-2.24458833390117));
#44248=CARTESIAN_POINT('Ctrl Pts',(-16.1933873263915,18.8965365797108,-2.24890449694883));
#44249=CARTESIAN_POINT('Ctrl Pts',(-16.2037176087823,18.8130761685129,-2.25308006086959));
#44250=CARTESIAN_POINT('Ctrl Pts',(-16.2181573115164,18.7301854648525,-2.25725562479036));
#44251=CARTESIAN_POINT('Ctrl Pts',(-16.236609460393,18.6482918228058,-2.26143118871113));
#44252=CARTESIAN_POINT('Ctrl Pts',(-16.2559935873462,18.5622619102622,-2.26581765132222));
#44253=CARTESIAN_POINT('Ctrl Pts',(-16.2798059943657,18.4773329921965,-2.27020411393331));
#44254=CARTESIAN_POINT('Ctrl Pts',(-16.3078756047626,18.3939807720539,-2.2745905765444));
#44255=CARTESIAN_POINT('Ctrl Pts',(-16.3359452151594,18.3106285519112,-2.2789770391555));
#44256=CARTESIAN_POINT('Ctrl Pts',(-16.3682717448907,18.2288535413147,-2.28336350176659));
#44257=CARTESIAN_POINT('Ctrl Pts',(-16.4046276535509,18.1491033611513,-2.28774996437768));
#44258=CARTESIAN_POINT('Ctrl Pts',(-16.4393107693519,18.0730226129128,-2.29193459890625));
#44259=CARTESIAN_POINT('Ctrl Pts',(-16.4777897133166,17.9985012713564,-2.29611923343482));
#44260=CARTESIAN_POINT('Ctrl Pts',(-16.5199018772185,17.9259437745003,-2.3003038679634));
#44261=CARTESIAN_POINT('Ctrl Pts',(-16.5619540996867,17.8534895542273,-2.30448254618457));
#44262=CARTESIAN_POINT('Ctrl Pts',(-16.6076290410406,17.7829940208021,-2.30866122440573));
#44263=CARTESIAN_POINT('Ctrl Pts',(-16.6567166746412,17.7148402537876,-2.3128399026269));
#44264=CARTESIAN_POINT('Ctrl Pts',(-16.7066841667541,17.6454648823148,-2.31709348047825));
#44265=CARTESIAN_POINT('Ctrl Pts',(-16.7601876992284,17.5785164938348,-2.32134705832959));
#44266=CARTESIAN_POINT('Ctrl Pts',(-16.8169575547354,17.5143715011666,-2.32560063618093));
#44267=CARTESIAN_POINT('Ctrl Pts',(-16.872626818136,17.4514700817286,-2.32977175029927));
#44268=CARTESIAN_POINT('Ctrl Pts',(-16.9314365679997,17.3912646900964,-2.33394286441762));
#44269=CARTESIAN_POINT('Ctrl Pts',(-16.9930907748647,17.3340782994918,-2.33811397853596));
#44270=CARTESIAN_POINT('Ctrl Pts',(-17.0547242930789,17.27691109832,-2.34228369299761));
#44271=CARTESIAN_POINT('Ctrl Pts',(-17.1192000356704,17.2227611988155,-2.34645340745925));
#44272=CARTESIAN_POINT('Ctrl Pts',(-17.1861855058205,17.1719143491242,-2.3506231219209));
#44273=CARTESIAN_POINT('Ctrl Pts',(-17.2531685923512,17.1210693087735,-2.35479268800691));
#44274=CARTESIAN_POINT('Ctrl Pts',(-17.3226608619368,17.0735273620081,-2.35896225409291));
#44275=CARTESIAN_POINT('Ctrl Pts',(-17.394298262154,17.0295327750314,-2.36313182017892));
#44276=CARTESIAN_POINT('Ctrl Pts',(-17.468454339619,16.9839913959473,-2.36744798275227));
#44277=CARTESIAN_POINT('Ctrl Pts',(-17.5449087501569,16.9422517437132,-2.37176414532562));
#44278=CARTESIAN_POINT('Ctrl Pts',(-17.6232285971903,16.9045336788281,-2.37608030789897));
#44279=CARTESIAN_POINT('Ctrl Pts',(-17.698997188932,16.8680442732967,-2.3802558722329));
#44280=CARTESIAN_POINT('Ctrl Pts',(-17.7765110982796,16.8353186125376,-2.38443143656682));
#44281=CARTESIAN_POINT('Ctrl Pts',(-17.855358497723,16.8065064752684,-2.38860700090075));
#44282=CARTESIAN_POINT('Ctrl Pts',(-17.938188283016,16.7762391086755,-2.39299346259381));
#44283=CARTESIAN_POINT('Ctrl Pts',(-18.022489249436,16.7502911703925,-2.39737992428687));
#44284=CARTESIAN_POINT('Ctrl Pts',(-18.1077688054804,16.7287763011746,-2.40176638597993));
#44285=CARTESIAN_POINT('Ctrl Pts',(-18.1930483615248,16.7072614319567,-2.40615284767299));
#44286=CARTESIAN_POINT('Ctrl Pts',(-18.2793059232537,16.6901796699007,-2.41053930936606));
#44287=CARTESIAN_POINT('Ctrl Pts',(-18.3660419494175,16.6775819782335,-2.41492577105912));
#44288=CARTESIAN_POINT('Ctrl Pts',(-18.4487871282915,16.6655639241848,-2.41911040544311));
#44289=CARTESIAN_POINT('Ctrl Pts',(-18.5322757027657,16.6575816378619,-2.42329503982711));
#44290=CARTESIAN_POINT('Ctrl Pts',(-18.6160795877536,16.6537173061283,-2.42747967421111));
#44291=CARTESIAN_POINT('Ctrl Pts',(-18.6997641882881,16.6498584747925,-2.43165835228622));
#44292=CARTESIAN_POINT('Ctrl Pts',(-18.7837627522533,16.6501059764733,-2.43583703036133));
#44293=CARTESIAN_POINT('Ctrl Pts',(-18.8676394869527,16.654490565727,-2.44001570843645));
#44294=CARTESIAN_POINT('Ctrl Pts',(-18.9530196520657,16.6589537456037,-2.44426928632412));
#44295=CARTESIAN_POINT('Ctrl Pts',(-19.0382731002408,16.6677038557804,-2.44852286421179));
#44296=CARTESIAN_POINT('Ctrl Pts',(-19.1229373349573,16.6807178518046,-2.45277644209946));
#44297=CARTESIAN_POINT('Ctrl Pts',(-19.2059601880682,16.6934795460894,-2.4569475560692));
#44298=CARTESIAN_POINT('Ctrl Pts',(-19.2884159943213,16.7103412009492,-2.46111867003895));
#44299=CARTESIAN_POINT('Ctrl Pts',(-19.369872949239,16.7312287217515,-2.46528978400869));
#44300=CARTESIAN_POINT('Ctrl Pts',(-19.4513025704935,16.7521092335458,-2.4694594983211));
#44301=CARTESIAN_POINT('Ctrl Pts',(-19.5317335608288,16.7770128141666,-2.47362921263351));
#44302=CARTESIAN_POINT('Ctrl Pts',(-19.6107456770747,16.8058145564779,-2.47779892694592));
#44303=CARTESIAN_POINT('Ctrl Pts',(-19.6897549817355,16.8346152739014,-2.48196849288227));
#44304=CARTESIAN_POINT('Ctrl Pts',(-19.7673450807723,16.867313718866,-2.48613805881862));
#44305=CARTESIAN_POINT('Ctrl Pts',(-19.8431135303122,16.9037359975767,-2.49030762475498));
#44306=CARTESIAN_POINT('Ctrl Pts',(-19.9215459053917,16.941438838831,-2.49462378750377));
#44307=CARTESIAN_POINT('Ctrl Pts',(-19.9980256738195,16.9831320175018,-2.49893995025257));
#44308=CARTESIAN_POINT('Ctrl Pts',(-20.0721336489296,17.0285705423537,-2.50325611300137));
#44309=CARTESIAN_POINT('Ctrl Pts',(-20.1438275642617,17.072528911864,-2.50743167718609));
#44310=CARTESIAN_POINT('Ctrl Pts',(-20.2133014733529,17.1199920607239,-2.51160724137082));
#44311=CARTESIAN_POINT('Ctrl Pts',(-20.2802065216066,17.1706947795633,-2.51578280555554));
#44312=CARTESIAN_POINT('Ctrl Pts',(-20.3504907852062,17.2239583725079,-2.52016926758637));
#44313=CARTESIAN_POINT('Ctrl Pts',(-20.4179394151737,17.2807970211654,-2.52455572961721));
#44314=CARTESIAN_POINT('Ctrl Pts',(-20.4821902270868,17.3408580455169,-2.52894219164805));
#44315=CARTESIAN_POINT('Ctrl Pts',(-20.546441039,17.4009190698683,-2.53332865367888));
#44316=CARTESIAN_POINT('Ctrl Pts',(-20.6074936847495,17.4642019995334,-2.53771511570972));
#44317=CARTESIAN_POINT('Ctrl Pts',(-20.665034920053,17.5303143846823,-2.54210157774055));
#44318=CARTESIAN_POINT('Ctrl Pts',(-20.7194682477108,17.5928559186633,-2.54625111891261));
#44319=CARTESIAN_POINT('Ctrl Pts',(-20.7709705307844,17.6581717364551,-2.55040066008466));
#44320=CARTESIAN_POINT('Ctrl Pts',(-20.8192426277969,17.7259534743927,-2.55455020125671));
#44321=CARTESIAN_POINT('Ctrl Pts',(-20.8674506257227,17.7936452069694,-2.55869423237604));
#44322=CARTESIAN_POINT('Ctrl Pts',(-20.912436679677,17.8637959851797,-2.56283826349536));
#44323=CARTESIAN_POINT('Ctrl Pts',(-20.953940279832,17.936062686255,-2.56698229461468));
#44324=CARTESIAN_POINT('Ctrl Pts',(-20.9954017278126,18.0082559913218,-2.57112211694435));
#44325=CARTESIAN_POINT('Ctrl Pts',(-21.0333875106824,18.0825605501461,-2.57526193927403));
#44326=CARTESIAN_POINT('Ctrl Pts',(-21.0676798966809,18.1586036203847,-2.5794017616037));
#44327=CARTESIAN_POINT('Ctrl Pts',(-21.1019481578681,18.2345931940623,-2.58353867155416));
#44328=CARTESIAN_POINT('Ctrl Pts',(-21.1325279904635,18.3123184247114,-2.58767558150461));
#44329=CARTESIAN_POINT('Ctrl Pts',(-21.1592478841653,18.3913825890383,-2.59181249145506));
#44330=CARTESIAN_POINT('Ctrl Pts',(-21.185962767493,18.4704319276684,-2.59594862567389));
#44331=CARTESIAN_POINT('Ctrl Pts',(-21.2088189905586,18.5508192612332,-2.60008475989273));
#44332=CARTESIAN_POINT('Ctrl Pts',(-21.2276938748212,18.6321296702378,-2.60422089411156));
#44333=CARTESIAN_POINT('Ctrl Pts',(-21.2465668271893,18.7134317569063,-2.60835660498608));
#44334=CARTESIAN_POINT('Ctrl Pts',(-21.261459151574,18.7956562735645,-2.61249231586059));
#44335=CARTESIAN_POINT('Ctrl Pts',(-21.272298987946,18.8783767179039,-2.61662802673511));
#44336=CARTESIAN_POINT('Ctrl Pts',(-21.2831447249188,18.9611421906275,-2.62076598885936));
#44337=CARTESIAN_POINT('Ctrl Pts',(-21.2899335186437,19.0444036643965,-2.62490395098361));
#44338=CARTESIAN_POINT('Ctrl Pts',(-21.2926453380231,19.1277291514849,-2.62904191310786));
#44339=CARTESIAN_POINT('Ctrl Pts',(-21.2935733586038,19.1562442389939,-2.63045797866241));
#44340=CARTESIAN_POINT('Ctrl Pts',(-21.2940243746441,19.1847668138181,-2.63187404421695));
#44341=CARTESIAN_POINT('Ctrl Pts',(-21.2939989850559,19.2132795861284,-2.6332901097715));
#44342=CARTESIAN_POINT('Ctrl Pts',(-21.2939989850552,19.2132795868247,-2.63329010980608));
#44343=CARTESIAN_POINT('Ctrl Pts',(-21.293907125607,19.3164386732131,-2.63841342883254));
#44344=CARTESIAN_POINT('Ctrl Pts',(-21.2875761055109,19.4193213099601,-2.643536747859));
#44345=CARTESIAN_POINT('Ctrl Pts',(-21.2751280763078,19.5212710102476,-2.64866006688546));
#44346=CARTESIAN_POINT('Ctrl Pts',(-21.2624749613816,19.6249003682273,-2.6538677944211));
#44347=CARTESIAN_POINT('Ctrl Pts',(-21.2435016684883,19.7275658815507,-2.65907552195674));
#44348=CARTESIAN_POINT('Ctrl Pts',(-21.2183850428165,19.8286009707164,-2.66428324949238));
#44349=CARTESIAN_POINT('Ctrl Pts',(-21.2103562166331,19.8608980308362,-2.66594796113558));
#44350=CARTESIAN_POINT('Ctrl Pts',(-21.2017000059957,19.8930286552932,-2.66761267277878));
#44351=CARTESIAN_POINT('Ctrl Pts',(-21.1924232051054,19.9249715292638,-2.66927738442198));
#44352=CARTESIAN_POINT('Ctrl Pts',(-21.1691038390111,20.0052672670978,-2.67346201883512));
#44353=CARTESIAN_POINT('Ctrl Pts',(-21.1418030734501,20.0845687630516,-2.67764665324825));
#44354=CARTESIAN_POINT('Ctrl Pts',(-21.1106233366689,20.1624523191421,-2.68183128766138));
#44355=CARTESIAN_POINT('Ctrl Pts',(-21.0794879803815,20.240225017636,-2.68600996576567));
#44356=CARTESIAN_POINT('Ctrl Pts',(-21.0444847892983,20.3165833617425,-2.69018864386997));
#44357=CARTESIAN_POINT('Ctrl Pts',(-21.0057661997906,20.3911179320259,-2.69436732197426));
#44358=CARTESIAN_POINT('Ctrl Pts',(-20.9663536076312,20.4669884804549,-2.69862089985464));
#44359=CARTESIAN_POINT('Ctrl Pts',(-20.923091244407,20.5409687666864,-2.70287447773502));
#44360=CARTESIAN_POINT('Ctrl Pts',(-20.8761915739271,20.6126473381688,-2.7071280556154));
#44361=CARTESIAN_POINT('Ctrl Pts',(-20.8302011447919,20.6829362811089,-2.71129916961421));
#44362=CARTESIAN_POINT('Ctrl Pts',(-20.7807134458812,20.7510115566354,-2.71547028361303));
#44363=CARTESIAN_POINT('Ctrl Pts',(-20.7279747027012,20.8165107863193,-2.71964139761184));
#44364=CARTESIAN_POINT('Ctrl Pts',(-20.675253656514,20.8819880371064,-2.72381111195321));
#44365=CARTESIAN_POINT('Ctrl Pts',(-20.6192840209111,20.944890600777,-2.72798082629459));
#44366=CARTESIAN_POINT('Ctrl Pts',(-20.560353487436,21.0048876606215,-2.73215054063596));
#44367=CARTESIAN_POINT('Ctrl Pts',(-20.5014250509605,21.064882585515,-2.73632010660112));
#44368=CARTESIAN_POINT('Ctrl Pts',(-20.4395362490684,21.1219718845495,-2.74048967256628));
#44369=CARTESIAN_POINT('Ctrl Pts',(-20.3750119946268,21.1758612249955,-2.74465923853145));
#44370=CARTESIAN_POINT('Ctrl Pts',(-20.3082191477172,21.2316452475716,-2.74897540124578));
#44371=CARTESIAN_POINT('Ctrl Pts',(-20.2386024799585,21.2839997657249,-2.75329156396011));
#44372=CARTESIAN_POINT('Ctrl Pts',(-20.1665585536104,21.3326446428367,-2.75760772667444));
#44373=CARTESIAN_POINT('Ctrl Pts',(-20.0968614498344,21.3797049187001,-2.76178329088732));
#44374=CARTESIAN_POINT('Ctrl Pts',(-20.0248932222208,21.4232933214429,-2.76595885510019));
#44375=CARTESIAN_POINT('Ctrl Pts',(-19.9510397173094,21.463202106049,-2.77013441931307));
#44376=CARTESIAN_POINT('Ctrl Pts',(-19.8734560486687,21.5051265878247,-2.77452088127813));
#44377=CARTESIAN_POINT('Ctrl Pts',(-19.7937921742969,21.5429897170771,-2.77890734324319));
#44378=CARTESIAN_POINT('Ctrl Pts',(-19.7125190809761,21.5766078305936,-2.78329380520824));
#44379=CARTESIAN_POINT('Ctrl Pts',(-19.6312459876554,21.61022594411,-2.7876802671733));
#44380=CARTESIAN_POINT('Ctrl Pts',(-19.5483642476832,21.6395989197709,-2.79206672913836));
#44381=CARTESIAN_POINT('Ctrl Pts',(-19.4643607861727,21.6646041086575,-2.79645319110342));
#44382=CARTESIAN_POINT('Ctrl Pts',(-19.3842194543331,21.6884596629912,-2.80063798179683));
#44383=CARTESIAN_POINT('Ctrl Pts',(-19.3027589678929,21.7084290356266,-2.80482277249024));
#44384=CARTESIAN_POINT('Ctrl Pts',(-19.2203910787649,21.7243689976798,-2.80900756318365));
#44385=CARTESIAN_POINT('Ctrl Pts',(-19.1381412613302,21.7402861103151,-2.81318635511555));
#44386=CARTESIAN_POINT('Ctrl Pts',(-19.0549870728557,21.7521851992274,-2.81736514704745));
#44387=CARTESIAN_POINT('Ctrl Pts',(-18.9713553167734,21.7599728232367,-2.82154393897936));
#44388=CARTESIAN_POINT('Ctrl Pts',(-18.8878237952947,21.7677511135976,-2.825717722532));
#44389=CARTESIAN_POINT('Ctrl Pts',(-18.8038162997617,21.771427693135,-2.82989150608464));
#44390=CARTESIAN_POINT('Ctrl Pts',(-18.7197682827693,21.7709604407538,-2.83406528963728));
#44391=CARTESIAN_POINT('Ctrl Pts',(-18.6357753750469,21.7704934947444,-2.83823633649044));
#44392=CARTESIAN_POINT('Ctrl Pts',(-18.5517424572939,21.7658881143933,-2.8424073833436));
#44393=CARTESIAN_POINT('Ctrl Pts',(-18.468107491185,21.7571541928477,-2.84657843019677));
#44394=CARTESIAN_POINT('Ctrl Pts',(-18.3845022745134,21.7484233780081,-2.85074799338464));
#44395=CARTESIAN_POINT('Ctrl Pts',(-18.3012951853464,21.7355669871492,-2.85491755657251));
#44396=CARTESIAN_POINT('Ctrl Pts',(-18.2189201971796,21.7186468644381,-2.85908711976038));
#44397=CARTESIAN_POINT('Ctrl Pts',(-18.1365498000665,21.7017276847462,-2.86325645056353));
#44398=CARTESIAN_POINT('Ctrl Pts',(-18.0550118619344,21.6807453176235,-2.86742578136668));
#44399=CARTESIAN_POINT('Ctrl Pts',(-17.9747299315205,21.655812664216,-2.87159511216983));
#44400=CARTESIAN_POINT('Ctrl Pts',(-17.8943836665539,21.6308600308318,-2.87576778409883));
#44401=CARTESIAN_POINT('Ctrl Pts',(-17.8152958594601,21.601950925752,-2.87994045602783));
#44402=CARTESIAN_POINT('Ctrl Pts',(-17.7378740400864,21.5692478817941,-2.88411312795683));
#44403=CARTESIAN_POINT('Ctrl Pts',(-17.6604189341951,21.5365307775821,-2.88828759387257));
#44404=CARTESIAN_POINT('Ctrl Pts',(-17.5846316581436,21.5000166836798,-2.89246205978831));
#44405=CARTESIAN_POINT('Ctrl Pts',(-17.510896867848,21.4599150113154,-2.89663652570405));
#44406=CARTESIAN_POINT('Ctrl Pts',(-17.4370550941973,21.4197551545928,-2.90081704844001));
#44407=CARTESIAN_POINT('Ctrl Pts',(-17.3652721469497,21.3759975630386,-2.90499757117598));
#44408=CARTESIAN_POINT('Ctrl Pts',(-17.2959049512236,21.3288958026033,-2.90917809391194));
#44409=CARTESIAN_POINT('Ctrl Pts',(-17.2545431057053,21.3008102541193,-2.91167083033844));
#44410=CARTESIAN_POINT('Ctrl Pts',(-17.2140395717351,21.2715365208939,-2.91416356676495));
#44411=CARTESIAN_POINT('Ctrl Pts',(-17.1744642439897,21.2411350264762,-2.91665630319145));
#44412=CARTESIAN_POINT('',(-21.2939990581246,19.2088040034447,-2.5667098902285));
#44413=CARTESIAN_POINT('Ctrl Pts',(-21.2953148853665,19.2088155456687,-2.56671052144854));
#44414=CARTESIAN_POINT('Ctrl Pts',(-21.2889869060013,19.9045867976347,-2.6013709944024));
#44415=CARTESIAN_POINT('Ctrl Pts',(-20.6359184624636,21.4617758669056,-2.67842340291674));
#44416=CARTESIAN_POINT('Ctrl Pts',(-18.5512406975192,22.0045420360256,-2.77291032223546));
#44417=CARTESIAN_POINT('Ctrl Pts',(-17.454631325708,21.4537986876689,-2.83273676860033));
#44418=CARTESIAN_POINT('Ctrl Pts',(-17.1767158522682,21.2382341403344,-2.85017127940472));
#44419=CARTESIAN_POINT('Ctrl Pts',(-17.1744642439897,21.2411350264762,-2.05017636798559));
#44420=CARTESIAN_POINT('Ctrl Pts',(-17.1080053551432,21.1900817654324,-2.054353901051));
#44421=CARTESIAN_POINT('Ctrl Pts',(-17.0439628152326,21.1356900431327,-2.05853143411641));
#44422=CARTESIAN_POINT('Ctrl Pts',(-16.9826883976904,21.0782192350166,-2.06270896718182));
#44423=CARTESIAN_POINT('Ctrl Pts',(-16.9214787266056,21.0208091542215,-2.06688208599938));
#44424=CARTESIAN_POINT('Ctrl Pts',(-16.863031698376,20.9603267674198,-2.07105520481693));
#44425=CARTESIAN_POINT('Ctrl Pts',(-16.8076662208124,20.8970718167269,-2.07522832363449));
#44426=CARTESIAN_POINT('Ctrl Pts',(-16.7523325270974,20.8338531790195,-2.07939904677548));
#44427=CARTESIAN_POINT('Ctrl Pts',(-16.7000771741035,20.7678654828481,-2.08356976991648));
#44428=CARTESIAN_POINT('Ctrl Pts',(-16.6511815739689,20.6994446258377,-2.08774049305747));
#44429=CARTESIAN_POINT('Ctrl Pts',(-16.6022993757804,20.6310425225115,-2.09191007303207));
#44430=CARTESIAN_POINT('Ctrl Pts',(-16.5567753686354,20.5602089570937,-2.09607965300666));
#44431=CARTESIAN_POINT('Ctrl Pts',(-16.5148492380406,20.4873110497425,-2.10024923298126));
#44432=CARTESIAN_POINT('Ctrl Pts',(-16.4729220223143,20.4144112556488,-2.10441892087286));
#44433=CARTESIAN_POINT('Ctrl Pts',(-16.4345930962794,20.3394474129684,-2.10858860876446));
#44434=CARTESIAN_POINT('Ctrl Pts',(-16.40005685324,20.2628124298998,-2.11275829665606));
#44435=CARTESIAN_POINT('Ctrl Pts',(-16.3654855176096,20.1860995773274,-2.11693222140548));
#44436=CARTESIAN_POINT('Ctrl Pts',(-16.3347147521372,20.1077126129561,-2.1211061461549));
#44437=CARTESIAN_POINT('Ctrl Pts',(-16.307891103021,20.028065248312,-2.12528007090433));
#44438=CARTESIAN_POINT('Ctrl Pts',(-16.281054150168,19.9483783809302,-2.129456065797));
#44439=CARTESIAN_POINT('Ctrl Pts',(-16.2581683384313,19.8674303112531,-2.13363206068967));
#44440=CARTESIAN_POINT('Ctrl Pts',(-16.2393298383502,19.7856484008281,-2.13780805558235));
#44441=CARTESIAN_POINT('Ctrl Pts',(-16.2204575688713,19.7037198903093,-2.14199153625323));
#44442=CARTESIAN_POINT('Ctrl Pts',(-16.2056471887002,19.6209550062764,-2.1461750169241));
#44443=CARTESIAN_POINT('Ctrl Pts',(-16.1949433808616,19.5377896644778,-2.15035849759498));
#44444=CARTESIAN_POINT('Ctrl Pts',(-16.1850243997655,19.4607221885294,-2.15423523625811));
#44445=CARTESIAN_POINT('Ctrl Pts',(-16.1786313156337,19.3833111752999,-2.15811197492124));
#44446=CARTESIAN_POINT('Ctrl Pts',(-16.175759706546,19.3059031134812,-2.16198871358438));
#44447=CARTESIAN_POINT('Ctrl Pts',(-16.1726600297933,19.222347182862,-2.16617334886855));
#44448=CARTESIAN_POINT('Ctrl Pts',(-16.1736524807725,19.1384837389767,-2.17035798415272));
#44449=CARTESIAN_POINT('Ctrl Pts',(-16.1787729918871,19.0547472015922,-2.17454261943689));
#44450=CARTESIAN_POINT('Ctrl Pts',(-16.1838862146021,18.9711298525711,-2.17872129842233));
#44451=CARTESIAN_POINT('Ctrl Pts',(-16.1931157984834,18.8876395064996,-2.18289997740777));
#44452=CARTESIAN_POINT('Ctrl Pts',(-16.2064457142957,18.8047127459324,-2.18707865639321));
#44453=CARTESIAN_POINT('Ctrl Pts',(-16.2200145556268,18.7202996054384,-2.19133223405457));
#44454=CARTESIAN_POINT('Ctrl Pts',(-16.2378321872334,18.6364709352134,-2.19558581171593));
#44455=CARTESIAN_POINT('Ctrl Pts',(-16.2598262335642,18.5536841143858,-2.19983938937729));
#44456=CARTESIAN_POINT('Ctrl Pts',(-16.2813938882842,18.4725022554353,-2.20401050427562));
#44457=CARTESIAN_POINT('Ctrl Pts',(-16.3069773455562,18.3923226754403,-2.20818161917395));
#44458=CARTESIAN_POINT('Ctrl Pts',(-16.3364567548607,18.3135667781462,-2.21235273407229));
#44459=CARTESIAN_POINT('Ctrl Pts',(-16.3659262721024,18.2348373080532,-2.21652244931808));
#44460=CARTESIAN_POINT('Ctrl Pts',(-16.3992889838848,18.157531002365,-2.22069216456387));
#44461=CARTESIAN_POINT('Ctrl Pts',(-16.4363757550798,18.0820523355112,-2.22486187980966));
#44462=CARTESIAN_POINT('Ctrl Pts',(-16.4734612066025,18.0065763544426,-2.22903144668293));
#44463=CARTESIAN_POINT('Ctrl Pts',(-16.5142702504276,17.9329282954129,-2.23320101355621));
#44464=CARTESIAN_POINT('Ctrl Pts',(-16.5585869493337,17.861489696597,-2.23737058042948));
#44465=CARTESIAN_POINT('Ctrl Pts',(-16.6044617469375,17.7875394398614,-2.24168674208251));
#44466=CARTESIAN_POINT('Ctrl Pts',(-16.6540951656361,17.7159573493129,-2.24600290373554));
#44467=CARTESIAN_POINT('Ctrl Pts',(-16.7071987883436,17.647134005604,-2.25031906538857));
#44468=CARTESIAN_POINT('Ctrl Pts',(-16.7585725904851,17.5805525435089,-2.25449463050951));
#44469=CARTESIAN_POINT('Ctrl Pts',(-16.8131936461488,17.5165531861027,-2.25867019563045));
#44470=CARTESIAN_POINT('Ctrl Pts',(-16.8707609575705,17.4554544236146,-2.26284576075139));
#44471=CARTESIAN_POINT('Ctrl Pts',(-16.9312358147182,17.3912697527985,-2.26723222067046));
#44472=CARTESIAN_POINT('Ctrl Pts',(-16.9949619538586,17.3302867948565,-2.27161868058953));
#44473=CARTESIAN_POINT('Ctrl Pts',(-17.0615499834747,17.2728279379207,-2.2760051405086));
#44474=CARTESIAN_POINT('Ctrl Pts',(-17.1281380130909,17.2153690809849,-2.28039160042767));
#44475=CARTESIAN_POINT('Ctrl Pts',(-17.1975874282728,17.1614346208606,-2.28477806034674));
#44476=CARTESIAN_POINT('Ctrl Pts',(-17.2694745299327,17.1112940330789,-2.28916452026581));
#44477=CARTESIAN_POINT('Ctrl Pts',(-17.3380540324817,17.0634604650508,-2.29334915467525));
#44478=CARTESIAN_POINT('Ctrl Pts',(-17.4091070955312,17.0189012759421,-2.29753378908469));
#44479=CARTESIAN_POINT('Ctrl Pts',(-17.4822878905536,16.977881822414,-2.30171842349413));
#44480=CARTESIAN_POINT('Ctrl Pts',(-17.5553645218218,16.9369207549729,-2.30589710159728));
#44481=CARTESIAN_POINT('Ctrl Pts',(-17.6305624715267,16.8994896383272,-2.31007577970044));
#44482=CARTESIAN_POINT('Ctrl Pts',(-17.707505966713,16.865811308311,-2.31425445780359));
#44483=CARTESIAN_POINT('Ctrl Pts',(-17.7858286183102,16.8315293186269,-2.31850803568458));
#44484=CARTESIAN_POINT('Ctrl Pts',(-17.8659596132368,16.8011362520549,-2.32276161356556));
#44485=CARTESIAN_POINT('Ctrl Pts',(-17.9474751923746,16.7748188230368,-2.32701519144655));
#44486=CARTESIAN_POINT('Ctrl Pts',(-18.027410433529,16.7490116085464,-2.33118630545055));
#44487=CARTESIAN_POINT('Ctrl Pts',(-18.1086765943189,16.7271235613587,-2.33535741945454));
#44488=CARTESIAN_POINT('Ctrl Pts',(-18.1908544682415,16.7092820040359,-2.33952853345854));
#44489=CARTESIAN_POINT('Ctrl Pts',(-18.2730047666345,16.6914464336092,-2.34369824780747));
#44490=CARTESIAN_POINT('Ctrl Pts',(-18.3560657213857,16.6776547538851,-2.34786796215639));
#44491=CARTESIAN_POINT('Ctrl Pts',(-18.4396056840353,16.667983683354,-2.35203767650532));
#44492=CARTESIAN_POINT('Ctrl Pts',(-18.5231426740242,16.6583129569554,-2.35620724248039));
#44493=CARTESIAN_POINT('Ctrl Pts',(-18.6071581809429,16.6527626002748,-2.36037680845547));
#44494=CARTESIAN_POINT('Ctrl Pts',(-18.6912145090002,16.6513575636898,-2.36454637443054));
#44495=CARTESIAN_POINT('Ctrl Pts',(-18.7782261526213,16.6499031277724,-2.36886253714027));
#44496=CARTESIAN_POINT('Ctrl Pts',(-18.8652810139811,16.6528909431617,-2.37317869984999));
#44497=CARTESIAN_POINT('Ctrl Pts',(-18.951894561366,16.6602899106078,-2.37749486255972));
#44498=CARTESIAN_POINT('Ctrl Pts',(-19.0356866828631,16.6674478575793,-2.38167042678835));
#44499=CARTESIAN_POINT('Ctrl Pts',(-19.1190653399936,16.6787338735463,-2.38584599101697));
#44500=CARTESIAN_POINT('Ctrl Pts',(-19.2015998086535,16.694067259749,-2.3900215552456));
#44501=CARTESIAN_POINT('Ctrl Pts',(-19.2883028951203,16.7101750984661,-2.39440801719588));
#44502=CARTESIAN_POINT('Ctrl Pts',(-19.3740737042673,16.7307497815343,-2.39879447914615));
#44503=CARTESIAN_POINT('Ctrl Pts',(-19.4584303876714,16.7556383945703,-2.40318094109643));
#44504=CARTESIAN_POINT('Ctrl Pts',(-19.5427870710755,16.7805270076064,-2.4075674030467));
#44505=CARTESIAN_POINT('Ctrl Pts',(-19.6257291067112,16.8097292861734,-2.41195386499698));
#44506=CARTESIAN_POINT('Ctrl Pts',(-19.7068005673283,16.8430348279154,-2.41634032694725));
#44507=CARTESIAN_POINT('Ctrl Pts',(-19.7841418063579,16.8748079308701,-2.42052496109111));
#44508=CARTESIAN_POINT('Ctrl Pts',(-19.8600687027665,16.9104332654798,-2.42470959523496));
#44509=CARTESIAN_POINT('Ctrl Pts',(-19.9341709431984,16.949763677299,-2.42889422937882));
#44510=CARTESIAN_POINT('Ctrl Pts',(-20.0081677081793,16.9890381071006,-2.43307290720919));
#44511=CARTESIAN_POINT('Ctrl Pts',(-20.0803445731189,17.0320069250119,-2.43725158503956));
#44512=CARTESIAN_POINT('Ctrl Pts',(-20.1503107695878,17.0784747823415,-2.44143026286993));
#44513=CARTESIAN_POINT('Ctrl Pts',(-20.2215310652186,17.125775546187,-2.44568384081822));
#44514=CARTESIAN_POINT('Ctrl Pts',(-20.290460214072,17.1767018411764,-2.4499374187665));
#44515=CARTESIAN_POINT('Ctrl Pts',(-20.3567118459902,17.2309984179595,-2.45419099671478));
#44516=CARTESIAN_POINT('Ctrl Pts',(-20.421679055696,17.2842423455132,-2.45836211043023));
#44517=CARTESIAN_POINT('Ctrl Pts',(-20.4840712680033,17.3407267365035,-2.46253322414569));
#44518=CARTESIAN_POINT('Ctrl Pts',(-20.5435545162614,17.4001680219639,-2.46670433786114));
#44519=CARTESIAN_POINT('Ctrl Pts',(-20.6030178043004,17.4595893612863,-2.47087405191626));
#44520=CARTESIAN_POINT('Ctrl Pts',(-20.6595737417694,17.5219652996142,-2.47504376597137));
#44521=CARTESIAN_POINT('Ctrl Pts',(-20.7129241774329,17.5869744152349,-2.47921348002649));
#44522=CARTESIAN_POINT('Ctrl Pts',(-20.7662727146278,17.6519812175144,-2.48338304570285));
#44523=CARTESIAN_POINT('Ctrl Pts',(-20.8164156856331,17.7196206546306,-2.48755261137921));
#44524=CARTESIAN_POINT('Ctrl Pts',(-20.863095194694,17.7895381989196,-2.49172217705558));
#44525=CARTESIAN_POINT('Ctrl Pts',(-20.9114159042677,17.8619139676384,-2.49603834010334));
#44526=CARTESIAN_POINT('Ctrl Pts',(-20.9560247758967,17.9367305826506,-2.5003545031511));
#44527=CARTESIAN_POINT('Ctrl Pts',(-20.9966856911894,18.0135637959011,-2.50467066619885));
#44528=CARTESIAN_POINT('Ctrl Pts',(-21.0360220760754,18.0878941651683,-2.50884623011952));
#44529=CARTESIAN_POINT('Ctrl Pts',(-21.0716636083121,18.1641113216876,-2.51302179404019));
#44530=CARTESIAN_POINT('Ctrl Pts',(-21.1034449999947,18.2418094139954,-2.51719735796086));
#44531=CARTESIAN_POINT('Ctrl Pts',(-21.1368316009424,18.3234318686752,-2.52158382057216));
#44532=CARTESIAN_POINT('Ctrl Pts',(-21.1659576673028,18.4066882444733,-2.52597028318347));
#44533=CARTESIAN_POINT('Ctrl Pts',(-21.1906909603742,18.491090613191,-2.53035674579477));
#44534=CARTESIAN_POINT('Ctrl Pts',(-21.2154242534456,18.5754929819087,-2.53474320840607));
#44535=CARTESIAN_POINT('Ctrl Pts',(-21.2357647130149,18.6610407614697,-2.53912967101737));
#44536=CARTESIAN_POINT('Ctrl Pts',(-21.251642469363,18.7472367021208,-2.54351613362868));
#44537=CARTESIAN_POINT('Ctrl Pts',(-21.2744558894944,18.8710844400873,-2.54981867488504));
#44538=CARTESIAN_POINT('Ctrl Pts',(-21.288135817693,18.9966631545043,-2.5561212161414));
#44539=CARTESIAN_POINT('Ctrl Pts',(-21.2924829866055,19.122881856295,-2.56242375739777));
#44540=CARTESIAN_POINT('Ctrl Pts',(-21.293468437957,19.1514941308042,-2.56385246834134));
#44541=CARTESIAN_POINT('Ctrl Pts',(-21.2939744691008,19.18013916897,-2.56528117928492));
#44542=CARTESIAN_POINT('Ctrl Pts',(-21.2939990581246,19.2088040034447,-2.5667098902285));
#44543=CARTESIAN_POINT('Origin',(-18.734,19.211,1.76670989022852));
#44544=CARTESIAN_POINT('',(-17.1744642439897,21.2411350264762,-1.25003885507116));
#44545=CARTESIAN_POINT('',(-17.1763037754664,21.2387764608408,-1.31677679026378));
#44546=CARTESIAN_POINT('',(-17.1744642439897,21.2411350264762,1.76670989022852));
#44547=CARTESIAN_POINT('',(-21.2937660440385,19.2099923323681,-1.83329006739986));
#44548=CARTESIAN_POINT('Ctrl Pts',(-17.1763037754663,21.2387764608407,-1.31677679026378));
#44549=CARTESIAN_POINT('Ctrl Pts',(-16.7482596486795,20.905321345112,-1.34369096604507));
#44550=CARTESIAN_POINT('Ctrl Pts',(-15.9020680777596,19.7058145697047,-1.41299707738683));
#44551=CARTESIAN_POINT('Ctrl Pts',(-16.4540142581906,17.2197793398558,-1.52469512428907));
#44552=CARTESIAN_POINT('Ctrl Pts',(-19.1741877306222,16.2160836252784,-1.65187093097051));
#44553=CARTESIAN_POINT('Ctrl Pts',(-21.0477248457009,17.6266607733557,-1.75473569409313));
#44554=CARTESIAN_POINT('Ctrl Pts',(-21.2914432046423,18.8451666090485,-1.81520852165527));
#44555=CARTESIAN_POINT('Ctrl Pts',(-21.2901594433486,19.2099805605233,-1.83328941365693));
#44556=CARTESIAN_POINT('Ctrl Pts',(-21.293999801981,19.2099930953476,-1.8332901097715));
#44557=CARTESIAN_POINT('Ctrl Pts',(-21.2940336318695,19.2960037294466,-1.83754657624536));
#44558=CARTESIAN_POINT('Ctrl Pts',(-21.289728450138,19.3819895209311,-1.84180304271922));
#44559=CARTESIAN_POINT('Ctrl Pts',(-21.2811180404437,19.4674950058893,-1.84605950919308));
#44560=CARTESIAN_POINT('Ctrl Pts',(-21.2725026284394,19.5530501661775,-1.85031844850686));
#44561=CARTESIAN_POINT('Ctrl Pts',(-21.2595770559904,19.6381240344265,-1.85457738782065));
#44562=CARTESIAN_POINT('Ctrl Pts',(-21.2424267246312,19.7222683905308,-1.85883632713443));
#44563=CARTESIAN_POINT('Ctrl Pts',(-21.2252479654662,19.8065522214573,-1.86310232592114));
#44564=CARTESIAN_POINT('Ctrl Pts',(-21.203830549429,19.8899030384947,-1.86736832470785));
#44565=CARTESIAN_POINT('Ctrl Pts',(-21.17831059956,19.9718848092049,-1.87163432349455));
#44566=CARTESIAN_POINT('Ctrl Pts',(-21.1527682031271,20.0539386885619,-1.87590407452273));
#44567=CARTESIAN_POINT('Ctrl Pts',(-21.1231162332672,20.1346207166622,-1.88017382555091));
#44568=CARTESIAN_POINT('Ctrl Pts',(-21.0895392515833,20.2135142563825,-1.88444357657908));
#44569=CARTESIAN_POINT('Ctrl Pts',(-21.0558918629605,20.2925732264768,-1.88872228076758));
#44570=CARTESIAN_POINT('Ctrl Pts',(-21.0183032080418,20.3698358258174,-1.89300098495607));
#44571=CARTESIAN_POINT('Ctrl Pts',(-20.9770042478451,20.4449092122797,-1.89727968914457));
#44572=CARTESIAN_POINT('Ctrl Pts',(-20.9482314695913,20.4972124637696,-1.90026064087417));
#44573=CARTESIAN_POINT('Ctrl Pts',(-20.9176587209492,20.5484536579338,-1.90324159260377));
#44574=CARTESIAN_POINT('Ctrl Pts',(-20.8853760800086,20.5985089053289,-1.90622254433338));
#44575=CARTESIAN_POINT('Ctrl Pts',(-20.8400579767351,20.6687760459572,-1.91040717961721));
#44576=CARTESIAN_POINT('Ctrl Pts',(-20.79120937469,20.7369513806192,-1.91459181490104));
#44577=CARTESIAN_POINT('Ctrl Pts',(-20.7390496454785,20.8026582293842,-1.91877645018487));
#44578=CARTESIAN_POINT('Ctrl Pts',(-20.6869641590402,20.8682715527659,-1.92295512916998));
#44579=CARTESIAN_POINT('Ctrl Pts',(-20.631577190453,20.9314230120947,-1.92713380815509));
#44580=CARTESIAN_POINT('Ctrl Pts',(-20.5731519436452,20.9917639170272,-1.9313124871402));
#44581=CARTESIAN_POINT('Ctrl Pts',(-20.5136794822353,21.0531863728336,-1.93556606480165));
#44582=CARTESIAN_POINT('Ctrl Pts',(-20.4510590119848,21.1116961211984,-1.93981964246309));
#44583=CARTESIAN_POINT('Ctrl Pts',(-20.3856118363234,21.1669596984898,-1.94407322012453));
#44584=CARTESIAN_POINT('Ctrl Pts',(-20.3214334643362,21.2211518983045,-1.94824433502252));
#44585=CARTESIAN_POINT('Ctrl Pts',(-20.2545373774524,21.2722223583836,-1.9524154499205));
#44586=CARTESIAN_POINT('Ctrl Pts',(-20.185263188972,21.3198942970985,-1.95658656481849));
#44587=CARTESIAN_POINT('Ctrl Pts',(-20.1160122460259,21.3675502390951,-1.96075628006393));
#44588=CARTESIAN_POINT('Ctrl Pts',(-20.0443851649613,21.4118096640091,-1.96492599530937));
#44589=CARTESIAN_POINT('Ctrl Pts',(-19.9707522614864,21.4524378964647,-1.96909571055481));
#44590=CARTESIAN_POINT('Ctrl Pts',(-19.8971219781182,21.493064683231,-1.97326527742773));
#44591=CARTESIAN_POINT('Ctrl Pts',(-19.8214864174479,21.5300603129431,-1.97743484430066));
#44592=CARTESIAN_POINT('Ctrl Pts',(-19.7442411220083,21.5632357185034,-1.98160441117358));
#44593=CARTESIAN_POINT('Ctrl Pts',(-19.6642800151965,21.5975775141097,-1.98592057282702));
#44594=CARTESIAN_POINT('Ctrl Pts',(-19.5825943571936,21.6278252448873,-1.99023673448046));
#44595=CARTESIAN_POINT('Ctrl Pts',(-19.4996442824009,21.653823946343,-1.99455289613389));
#44596=CARTESIAN_POINT('Ctrl Pts',(-19.4193962595357,21.6789757547542,-1.99872846125448));
#44597=CARTESIAN_POINT('Ctrl Pts',(-19.337965398231,21.7001510303436,-2.00290402637506));
#44598=CARTESIAN_POINT('Ctrl Pts',(-19.2557808536486,21.7172611078588,-2.00707959149565));
#44599=CARTESIAN_POINT('Ctrl Pts',(-19.1694454234896,21.7352353621403,-2.01146605141551));
#44600=CARTESIAN_POINT('Ctrl Pts',(-19.0822787502277,21.7487228765315,-2.01585251133537));
#44601=CARTESIAN_POINT('Ctrl Pts',(-18.9947846789879,21.7576824205631,-2.02023897125523));
#44602=CARTESIAN_POINT('Ctrl Pts',(-18.9072906077481,21.7666419645947,-2.02462543117509));
#44603=CARTESIAN_POINT('Ctrl Pts',(-18.8194697218412,21.7710735849931,-2.02901189109496));
#44604=CARTESIAN_POINT('Ctrl Pts',(-18.7318236815475,21.7709990749291,-2.03339835101482));
#44605=CARTESIAN_POINT('Ctrl Pts',(-18.6482254298112,21.7709280059902,-2.03758222948078));
#44606=CARTESIAN_POINT('Ctrl Pts',(-18.5644751184015,21.7667575762838,-2.04176610794674));
#44607=CARTESIAN_POINT('Ctrl Pts',(-18.4810079806566,21.7584683586158,-2.04594998641271));
#44608=CARTESIAN_POINT('Ctrl Pts',(-18.3976520608152,21.750190186126,-2.05012828996374));
#44609=CARTESIAN_POINT('Ctrl Pts',(-18.3145790190074,21.7378041671174,-2.05430659351478));
#44610=CARTESIAN_POINT('Ctrl Pts',(-18.23222439898,21.7213428543171,-2.05848489706582));
#44611=CARTESIAN_POINT('Ctrl Pts',(-18.1499547981595,21.704898535436,-2.06265888712414));
#44612=CARTESIAN_POINT('Ctrl Pts',(-18.0684025946749,21.6843873684699,-2.06683287718245));
#44613=CARTESIAN_POINT('Ctrl Pts',(-17.987997155172,21.6598935778242,-2.07100686724077));
#44614=CARTESIAN_POINT('Ctrl Pts',(-17.9076457851309,21.635416258279,-2.0751780504567));
#44615=CARTESIAN_POINT('Ctrl Pts',(-17.8284400864338,21.6069617675245,-2.07934923367263));
#44616=CARTESIAN_POINT('Ctrl Pts',(-17.7507969266643,21.5746648909232,-2.08352041688856));
#44617=CARTESIAN_POINT('Ctrl Pts',(-17.6731854101502,21.5423811768249,-2.08768990015028));
#44618=CARTESIAN_POINT('Ctrl Pts',(-17.5971355905954,21.506258367263,-2.09185938341201));
#44619=CARTESIAN_POINT('Ctrl Pts',(-17.5230455881588,21.4664798630097,-2.09602886667374));
#44620=CARTESIAN_POINT('Ctrl Pts',(-17.4489417854745,21.4266939494813,-2.10019912655714));
#44621=CARTESIAN_POINT('Ctrl Pts',(-17.3767989370809,21.3832511941844,-2.10436938644054));
#44622=CARTESIAN_POINT('Ctrl Pts',(-17.3069908375595,21.3363811070749,-2.10853964632394));
#44623=CARTESIAN_POINT('Ctrl Pts',(-17.2618060884471,21.3060434651473,-2.11123893405498));
#44624=CARTESIAN_POINT('Ctrl Pts',(-17.2175989879755,21.274270839954,-2.11393822178602));
#44625=CARTESIAN_POINT('Ctrl Pts',(-17.1744642439897,21.2411350264762,-2.11663750951706));
#44626=CARTESIAN_POINT('',(-21.2939995273705,19.2125555907563,-1.76670989019937));
#44627=CARTESIAN_POINT('Ctrl Pts',(-21.2939995273702,19.2125555913393,-1.7667098902285));
#44628=CARTESIAN_POINT('Ctrl Pts',(-21.2939437779102,19.3043011465908,-1.77129369133236));
#44629=CARTESIAN_POINT('Ctrl Pts',(-21.2889563823285,19.3958958079181,-1.77587749243622));
#44630=CARTESIAN_POINT('Ctrl Pts',(-21.2790836672346,19.4869513123279,-1.78046129354008));
#44631=CARTESIAN_POINT('Ctrl Pts',(-21.2700706759975,19.5700776312323,-1.78464593361015));
#44632=CARTESIAN_POINT('Ctrl Pts',(-21.2569640809886,19.6529166096931,-1.78883057368023));
#44633=CARTESIAN_POINT('Ctrl Pts',(-21.2397911343996,19.7350331962428,-1.7930152137503));
#44634=CARTESIAN_POINT('Ctrl Pts',(-21.2226426310956,19.817032901329,-1.79719389757114));
#44635=CARTESIAN_POINT('Ctrl Pts',(-21.2014393661311,19.8983118104412,-1.80137258139199));
#44636=CARTESIAN_POINT('Ctrl Pts',(-21.1762603200948,19.9784402445079,-1.80555126521283));
#44637=CARTESIAN_POINT('Ctrl Pts',(-21.150630001539,20.0600047838296,-1.80980484167153));
#44638=CARTESIAN_POINT('Ctrl Pts',(-21.1208800342882,20.1403767226468,-1.81405841813022));
#44639=CARTESIAN_POINT('Ctrl Pts',(-21.0871481593181,20.21911395204,-1.81831199458892));
#44640=CARTESIAN_POINT('Ctrl Pts',(-21.0540701851445,20.2963248406336,-1.82248311440869));
#44641=CARTESIAN_POINT('Ctrl Pts',(-21.0171634957605,20.3719633904436,-1.82665423422847));
#44642=CARTESIAN_POINT('Ctrl Pts',(-20.9766076076857,20.4456299518278,-1.83082535404824));
#44643=CARTESIAN_POINT('Ctrl Pts',(-20.9360653282555,20.5192717941858,-1.83499507423679));
#44644=CARTESIAN_POINT('Ctrl Pts',(-20.8918765036875,20.5909425596168,-1.83916479442534));
#44645=CARTESIAN_POINT('Ctrl Pts',(-20.8442669697396,20.6602664752991,-1.84333451461389));
#44646=CARTESIAN_POINT('Ctrl Pts',(-20.7966591297285,20.7295879244518,-1.84750408644471));
#44647=CARTESIAN_POINT('Ctrl Pts',(-20.7456310834599,20.7965623111441,-1.85167365827553));
#44648=CARTESIAN_POINT('Ctrl Pts',(-20.691451661047,20.8608433242779,-1.85584323010635));
#44649=CARTESIAN_POINT('Ctrl Pts',(-20.6353675257683,20.9273841782754,-1.86015938594928));
#44650=CARTESIAN_POINT('Ctrl Pts',(-20.5759066466623,20.9910383508709,-1.86447554179221));
#44651=CARTESIAN_POINT('Ctrl Pts',(-20.5134108769448,21.0514610647907,-1.86879169763514));
#44652=CARTESIAN_POINT('Ctrl Pts',(-20.4529507187175,21.1099156907698,-1.87296726769975));
#44653=CARTESIAN_POINT('Ctrl Pts',(-20.3896507250023,21.1653458615584,-1.87714283776436));
#44654=CARTESIAN_POINT('Ctrl Pts',(-20.3238547775404,21.2174799491478,-1.88131840782897));
#44655=CARTESIAN_POINT('Ctrl Pts',(-20.2547359396678,21.2722469627211,-1.88570485656106));
#44656=CARTESIAN_POINT('Ctrl Pts',(-20.1828628806314,21.3233758659983,-1.89009130529315));
#44657=CARTESIAN_POINT('Ctrl Pts',(-20.1086675060193,21.3706039562602,-1.89447775402525));
#44658=CARTESIAN_POINT('Ctrl Pts',(-20.0344721314073,21.417832046522,-1.89886420275734));
#44659=CARTESIAN_POINT('Ctrl Pts',(-19.9579549835793,21.4611591040721,-1.90325065148943));
#44660=CARTESIAN_POINT('Ctrl Pts',(-19.8795742651121,21.5003797420072,-1.90763710022152));
#44661=CARTESIAN_POINT('Ctrl Pts',(-19.8047997208671,21.5377958997554,-1.91182173531048));
#44662=CARTESIAN_POINT('Ctrl Pts',(-19.7280509965254,21.5716144630821,-1.91600637039945));
#44663=CARTESIAN_POINT('Ctrl Pts',(-19.6497086514407,21.6016228614477,-1.92019100548841));
#44664=CARTESIAN_POINT('Ctrl Pts',(-19.5714778164362,21.6315885467837,-1.92436968429672));
#44665=CARTESIAN_POINT('Ctrl Pts',(-19.4916582921888,21.6577546763365,-1.92854836310503));
#44666=CARTESIAN_POINT('Ctrl Pts',(-19.4106541204074,21.6799550828915,-1.93272704191334));
#44667=CARTESIAN_POINT('Ctrl Pts',(-19.3281980247988,21.7025534109181,-1.93698061962124));
#44668=CARTESIAN_POINT('Ctrl Pts',(-19.2445148260133,21.7210422324063,-1.94123419732914));
#44669=CARTESIAN_POINT('Ctrl Pts',(-19.1600508252197,21.7352980597246,-1.94548777503704));
#44670=CARTESIAN_POINT('Ctrl Pts',(-19.0772243047676,21.7492775132415,-1.94965888980438));
#44671=CARTESIAN_POINT('Ctrl Pts',(-18.9936474610422,21.7591865556584,-1.95383000457171));
#44672=CARTESIAN_POINT('Ctrl Pts',(-18.9097535041071,21.7649598089622,-1.95800111933905));
#44673=CARTESIAN_POINT('Ctrl Pts',(-18.8258876981392,21.7707311250267,-1.96217083447142));
#44674=CARTESIAN_POINT('Ctrl Pts',(-18.7417054488562,21.7723693765771,-1.9663405496038));
#44675=CARTESIAN_POINT('Ctrl Pts',(-18.6576449614605,21.769861056816,-1.97051026473618));
#44676=CARTESIAN_POINT('Ctrl Pts',(-18.573587464861,21.7673528262987,-1.97467983151386));
#44677=CARTESIAN_POINT('Ctrl Pts',(-18.489652181338,21.7606983323727,-1.97884939829155));
#44678=CARTESIAN_POINT('Ctrl Pts',(-18.4062758155004,21.7499361667624,-1.98301896506923));
#44679=CARTESIAN_POINT('Ctrl Pts',(-18.3199680751373,21.7387956212864,-1.9873351268887));
#44680=CARTESIAN_POINT('Ctrl Pts',(-18.2342598094106,21.7232532494571,-1.99165128870818));
#44681=CARTESIAN_POINT('Ctrl Pts',(-18.149625962838,21.7034098749385,-1.99596745052766));
#44682=CARTESIAN_POINT('Ctrl Pts',(-18.0677490202284,21.6842128881249,-2.00014301559882));
#44683=CARTESIAN_POINT('Ctrl Pts',(-17.9868780138841,21.6609909777852,-2.00431858066999));
#44684=CARTESIAN_POINT('Ctrl Pts',(-17.9074274757339,21.6338862668578,-2.00849414574115));
#44685=CARTESIAN_POINT('Ctrl Pts',(-17.8239641319665,21.6054125792212,-2.01288060593478));
#44686=CARTESIAN_POINT('Ctrl Pts',(-17.7420690633811,21.5726537644299,-2.01726706612842));
#44687=CARTESIAN_POINT('Ctrl Pts',(-17.6621969477251,21.5358307932265,-2.02165352632205));
#44688=CARTESIAN_POINT('Ctrl Pts',(-17.5823248320691,21.4990078220231,-2.02603998651568));
#44689=CARTESIAN_POINT('Ctrl Pts',(-17.5044761476508,21.458121031537,-2.03042644670931));
#44690=CARTESIAN_POINT('Ctrl Pts',(-17.4290716121317,21.4134445288214,-2.03481290690294));
#44691=CARTESIAN_POINT('Ctrl Pts',(-17.3571349231711,21.370822693708,-2.03899763425939));
#44692=CARTESIAN_POINT('Ctrl Pts',(-17.2871547392091,21.3245934161538,-2.04318236161584));
#44693=CARTESIAN_POINT('Ctrl Pts',(-17.2195158137623,21.2749616395747,-2.0473670889723));
#44694=CARTESIAN_POINT('Ctrl Pts',(-17.2043800914437,21.2638554195465,-2.04830351531006));
#44695=CARTESIAN_POINT('Ctrl Pts',(-17.1893615177922,21.2525790096887,-2.04923994164783));
#44696=CARTESIAN_POINT('Ctrl Pts',(-17.1744642439897,21.2411350264762,-2.05017636798559));
#44697=CARTESIAN_POINT('Ctrl Pts',(-17.1744642439897,21.2411350264762,-1.25003885507116));
#44698=CARTESIAN_POINT('Ctrl Pts',(-17.1078166447992,21.1899367994448,-1.25422272222311));
#44699=CARTESIAN_POINT('Ctrl Pts',(-17.0437743697779,21.1355158045555,-1.25840658937506));
#44700=CARTESIAN_POINT('Ctrl Pts',(-16.9826476100414,21.0781809784234,-1.26259045652701));
#44701=CARTESIAN_POINT('Ctrl Pts',(-16.9380010114888,21.0363039841833,-1.26564632662279));
#44702=CARTESIAN_POINT('Ctrl Pts',(-16.8949090211694,20.9928733428054,-1.26870219671856));
#44703=CARTESIAN_POINT('Ctrl Pts',(-16.8534788428352,20.9480204884962,-1.27175806681434));
#44704=CARTESIAN_POINT('Ctrl Pts',(-16.7967467984314,20.8866016333375,-1.27594259521698));
#44705=CARTESIAN_POINT('Ctrl Pts',(-16.7429212490902,20.8222861496523,-1.28012712361962));
#44706=CARTESIAN_POINT('Ctrl Pts',(-16.6923122077178,20.755380444983,-1.28431165202226));
#44707=CARTESIAN_POINT('Ctrl Pts',(-16.6417752234727,20.6885700006218,-1.2884902224955));
#44708=CARTESIAN_POINT('Ctrl Pts',(-16.5944459257277,20.6191770244766,-1.29266879296874));
#44709=CARTESIAN_POINT('Ctrl Pts',(-16.5505962863687,20.5475433862397,-1.29684736344198));
#44710=CARTESIAN_POINT('Ctrl Pts',(-16.5059592440482,20.4746234309494,-1.30110096802756));
#44711=CARTESIAN_POINT('Ctrl Pts',(-16.464928391305,20.3993819010163,-1.30535457261313));
#44712=CARTESIAN_POINT('Ctrl Pts',(-16.4277464801527,20.322213166855,-1.30960817719871));
#44713=CARTESIAN_POINT('Ctrl Pts',(-16.3912866103988,20.2465429845162,-1.3137791803658));
#44714=CARTESIAN_POINT('Ctrl Pts',(-16.3585277410935,20.1690202117746,-1.3179501835329));
#44715=CARTESIAN_POINT('Ctrl Pts',(-16.3296531424777,20.0900427684264,-1.32212118669999));
#44716=CARTESIAN_POINT('Ctrl Pts',(-16.3007882398715,20.011091845483,-1.32629078925587));
#44717=CARTESIAN_POINT('Ctrl Pts',(-16.2758051753869,19.9306876537765,-1.33046039181176));
#44718=CARTESIAN_POINT('Ctrl Pts',(-16.2548387836586,19.8492473371574,-1.33462999436764));
#44719=CARTESIAN_POINT('Ctrl Pts',(-16.2338731420879,19.7678099343954,-1.3387994477391));
#44720=CARTESIAN_POINT('Ctrl Pts',(-16.2169240014122,19.6853369261728,-1.34296890111057));
#44721=CARTESIAN_POINT('Ctrl Pts',(-16.2040757356768,19.6022585037906,-1.34713835448203));
#44722=CARTESIAN_POINT('Ctrl Pts',(-16.1907749795004,19.5162542241174,-1.35145464773318));
#44723=CARTESIAN_POINT('Ctrl Pts',(-16.1818694215614,19.4296016124723,-1.35577094098433));
#44724=CARTESIAN_POINT('Ctrl Pts',(-16.1773942973163,19.3427849801953,-1.36008723423547));
#44725=CARTESIAN_POINT('Ctrl Pts',(-16.1730651983007,19.2588012119818,-1.36426268498078));
#44726=CARTESIAN_POINT('Ctrl Pts',(-16.1728818000995,19.1746644338097,-1.36843813572608));
#44727=CARTESIAN_POINT('Ctrl Pts',(-16.1768228602554,19.0908123302178,-1.37261358647139));
#44728=CARTESIAN_POINT('Ctrl Pts',(-16.1809633247949,19.0027175923176,-1.37700030097545));
#44729=CARTESIAN_POINT('Ctrl Pts',(-16.1896565650922,18.9149376772192,-1.38138701547952));
#44730=CARTESIAN_POINT('Ctrl Pts',(-16.2028167402278,18.8279708817217,-1.38577372998358));
#44731=CARTESIAN_POINT('Ctrl Pts',(-16.2159769153634,18.7410040862241,-1.39016044448765));
#44732=CARTESIAN_POINT('Ctrl Pts',(-16.2336038344097,18.6548509637837,-1.39454715899172));
#44733=CARTESIAN_POINT('Ctrl Pts',(-16.2555511520629,18.5699919593647,-1.39893387349578));
#44734=CARTESIAN_POINT('Ctrl Pts',(-16.2764876099038,18.489041430625,-1.40311854265335));
#44735=CARTESIAN_POINT('Ctrl Pts',(-16.3014331762482,18.4089670881459,-1.40730321181092));
#44736=CARTESIAN_POINT('Ctrl Pts',(-16.3302979817924,18.3301954770413,-1.41148788096849));
#44737=CARTESIAN_POINT('Ctrl Pts',(-16.3591217043841,18.2515359806832,-1.41566659413361));
#44738=CARTESIAN_POINT('Ctrl Pts',(-16.3918534291669,18.1741759609909,-1.41984530729872));
#44739=CARTESIAN_POINT('Ctrl Pts',(-16.4283528787703,18.0985291678587,-1.42402402046383));
#44740=CARTESIAN_POINT('Ctrl Pts',(-16.4655061666039,18.0215272648309,-1.42827758961855));
#44741=CARTESIAN_POINT('Ctrl Pts',(-16.5065633783675,17.9463010412761,-1.43253115877328));
#44742=CARTESIAN_POINT('Ctrl Pts',(-16.5513243019902,17.8732680398086,-1.436784727928));
#44743=CARTESIAN_POINT('Ctrl Pts',(-16.5952179124827,17.8016501673418,-1.44095587750601));
#44744=CARTESIAN_POINT('Ctrl Pts',(-16.6426727330391,17.7321416910373,-1.44512702708403));
#44745=CARTESIAN_POINT('Ctrl Pts',(-16.6934533489152,17.6651121111974,-1.44929817666204));
#44746=CARTESIAN_POINT('Ctrl Pts',(-16.7442169264156,17.598105021734,-1.45346792669788));
#44747=CARTESIAN_POINT('Ctrl Pts',(-16.7983038054767,17.5335755432561,-1.45763767673371));
#44748=CARTESIAN_POINT('Ctrl Pts',(-16.8554361909196,17.4718628532479,-1.46180742676954));
#44749=CARTESIAN_POINT('Ctrl Pts',(-16.9125665442965,17.4101523582163,-1.46597702849708));
#44750=CARTESIAN_POINT('Ctrl Pts',(-16.9727418755408,17.3512587894506,-1.47014663022461));
#44751=CARTESIAN_POINT('Ctrl Pts',(-17.0356461063899,17.2954859561832,-1.47431623195215));
#44752=CARTESIAN_POINT('Ctrl Pts',(-17.1007607791355,17.237753276882,-1.47863235263757));
#44753=CARTESIAN_POINT('Ctrl Pts',(-17.1687993162101,17.1833650934407,-1.48294847332299));
#44754=CARTESIAN_POINT('Ctrl Pts',(-17.2393736228791,17.1326131272512,-1.48726459400841));
#44755=CARTESIAN_POINT('Ctrl Pts',(-17.3076502260402,17.0835135041913,-1.49144019378605));
#44756=CARTESIAN_POINT('Ctrl Pts',(-17.3782995960785,17.0378171774819,-1.49561579356368));
#44757=CARTESIAN_POINT('Ctrl Pts',(-17.4509421894257,16.9957432079499,-1.49979139334132));
#44758=CARTESIAN_POINT('Ctrl Pts',(-17.5272517301713,16.9515453738088,-1.50417777448063));
#44759=CARTESIAN_POINT('Ctrl Pts',(-17.6057605029808,16.9113454944654,-1.50856415561995));
#44760=CARTESIAN_POINT('Ctrl Pts',(-17.6860031863916,16.8753410611421,-1.51295053675926));
#44761=CARTESIAN_POINT('Ctrl Pts',(-17.7662458698024,16.8393366278189,-1.51733691789858));
#44762=CARTESIAN_POINT('Ctrl Pts',(-17.8482218954648,16.8075277794807,-1.52172329903789));
#44763=CARTESIAN_POINT('Ctrl Pts',(-17.9314482086486,16.7800514974195,-1.52610968017721));
#44764=CARTESIAN_POINT('Ctrl Pts',(-18.0108467907137,16.7538389000734,-1.53029432358547));
#44765=CARTESIAN_POINT('Ctrl Pts',(-18.0916786884036,16.7314715385808,-1.53447896699374));
#44766=CARTESIAN_POINT('Ctrl Pts',(-18.1735366057567,16.7131047292344,-1.538663610402));
#44767=CARTESIAN_POINT('Ctrl Pts',(-18.2552780138067,16.6947640615763,-1.5428422977598));
#44768=CARTESIAN_POINT('Ctrl Pts',(-18.3380420957822,16.6804127357782,-1.5470209851176));
#44769=CARTESIAN_POINT('Ctrl Pts',(-18.421405029143,16.6701567572566,-1.5511996724754));
#44770=CARTESIAN_POINT('Ctrl Pts',(-18.5062619492397,16.6597169764711,-1.5554532480747));
#44771=CARTESIAN_POINT('Ctrl Pts',(-18.5917389394536,16.6535209329784,-1.559706823674));
#44772=CARTESIAN_POINT('Ctrl Pts',(-18.6773765359446,16.651626290805,-1.5639603992733));
#44773=CARTESIAN_POINT('Ctrl Pts',(-18.7613541238536,16.6497683745839,-1.56813152309571));
#44774=CARTESIAN_POINT('Ctrl Pts',(-18.8454856660802,16.6520466005361,-1.57230264691812));
#44775=CARTESIAN_POINT('Ctrl Pts',(-18.9293330503143,16.6584630268192,-1.57647377074053));
#44776=CARTESIAN_POINT('Ctrl Pts',(-19.0131523026761,16.6648773003091,-1.58064349509743));
#44777=CARTESIAN_POINT('Ctrl Pts',(-19.0966871280817,16.6754269816346,-1.58481321945433));
#44778=CARTESIAN_POINT('Ctrl Pts',(-19.1795019710685,16.6900620805395,-1.58898294381123));
#44779=CARTESIAN_POINT('Ctrl Pts',(-19.2623138707192,16.7046966592958,-1.59315251997126));
#44780=CARTESIAN_POINT('Ctrl Pts',(-19.3444053859658,16.7234162860397,-1.59732209613129));
#44781=CARTESIAN_POINT('Ctrl Pts',(-19.4253499785112,16.7461196363287,-1.60149167229132));
#44782=CARTESIAN_POINT('Ctrl Pts',(-19.5091400540413,16.7696210880709,-1.60580782350526));
#44783=CARTESIAN_POINT('Ctrl Pts',(-19.5917005594529,16.7973914247812,-1.6101239747192));
#44784=CARTESIAN_POINT('Ctrl Pts',(-19.6725761219549,16.8292622177712,-1.61444012593315));
#44785=CARTESIAN_POINT('Ctrl Pts',(-19.7508175783492,16.8600949833538,-1.61861570068712));
#44786=CARTESIAN_POINT('Ctrl Pts',(-19.8274817539353,16.8947649658156,-1.62279127544109));
#44787=CARTESIAN_POINT('Ctrl Pts',(-19.9021790183312,16.9330716031599,-1.62696685019507));
#44788=CARTESIAN_POINT('Ctrl Pts',(-19.9806484617505,16.9733127088547,-1.631353289639));
#44789=CARTESIAN_POINT('Ctrl Pts',(-20.0569466030573,17.0175671444772,-1.63573972908293));
#44790=CARTESIAN_POINT('Ctrl Pts',(-20.130655495903,17.0655505305965,-1.64012616852686));
#44791=CARTESIAN_POINT('Ctrl Pts',(-20.2043643887487,17.1135339167158,-1.64451260797079));
#44792=CARTESIAN_POINT('Ctrl Pts',(-20.275483608608,17.1652458506084,-1.64889904741472));
#44793=CARTESIAN_POINT('Ctrl Pts',(-20.3436364934689,17.2203542859431,-1.65328548685865));
#44794=CARTESIAN_POINT('Ctrl Pts',(-20.4078056279229,17.2722414599601,-1.6574155251252));
#44795=CARTESIAN_POINT('Ctrl Pts',(-20.4695977832764,17.3273436084189,-1.66154556339175));
#44796=CARTESIAN_POINT('Ctrl Pts',(-20.5286666498128,17.3854119807444,-1.6656756016583));
#44797=CARTESIAN_POINT('Ctrl Pts',(-20.5888757459544,17.4446012697411,-1.66988536368084));
#44798=CARTESIAN_POINT('Ctrl Pts',(-20.6462548736576,17.5068722657662,-1.67409512570339));
#44799=CARTESIAN_POINT('Ctrl Pts',(-20.7004701683271,17.5719163910649,-1.67830488772593));
#44800=CARTESIAN_POINT('Ctrl Pts',(-20.7535207653518,17.6355631848541,-1.68242421217099));
#44801=CARTESIAN_POINT('Ctrl Pts',(-20.8035417767949,17.7018647731871,-1.68654353661605));
#44802=CARTESIAN_POINT('Ctrl Pts',(-20.850256855771,17.7704942136866,-1.69066286106111));
#44803=CARTESIAN_POINT('Ctrl Pts',(-20.8969436374088,17.8390820823739,-1.69477969025368));
#44804=CARTESIAN_POINT('Ctrl Pts',(-20.9403281944971,17.9099946152069,-1.69889651944625));
#44805=CARTESIAN_POINT('Ctrl Pts',(-20.9801755816481,17.9828732734739,-1.70301334863882));
#44806=CARTESIAN_POINT('Ctrl Pts',(-21.0200115244872,18.05573100073,-1.70712899546334));
#44807=CARTESIAN_POINT('Ctrl Pts',(-21.0563120879347,18.1305533171676,-1.71124464228787));
#44808=CARTESIAN_POINT('Ctrl Pts',(-21.088887451558,18.206955633204,-1.71536028911239));
#44809=CARTESIAN_POINT('Ctrl Pts',(-21.1227568123705,18.2863928925596,-1.71963942253631));
#44810=CARTESIAN_POINT('Ctrl Pts',(-21.1525985841264,18.3675378137456,-1.72391855596022));
#44811=CARTESIAN_POINT('Ctrl Pts',(-21.1782545843983,18.4499352677678,-1.72819768938414));
#44812=CARTESIAN_POINT('Ctrl Pts',(-21.2029529680662,18.5292572162836,-1.73231710308656));
#44813=CARTESIAN_POINT('Ctrl Pts',(-21.2237724320015,18.6097393655103,-1.73643651678898));
#44814=CARTESIAN_POINT('Ctrl Pts',(-21.2406233770012,18.6909622649548,-1.7405559304914));
#44815=CARTESIAN_POINT('Ctrl Pts',(-21.2574836176246,18.7722299700469,-1.74467761661945));
#44816=CARTESIAN_POINT('Ctrl Pts',(-21.2703709121366,18.8542387712825,-1.74879930274751));
#44817=CARTESIAN_POINT('Ctrl Pts',(-21.279247341302,18.9365624449985,-1.75292098887556));
#44818=CARTESIAN_POINT('Ctrl Pts',(-21.2881358451795,19.0189981045868,-1.75704828178227));
#44819=CARTESIAN_POINT('Ctrl Pts',(-21.2930025796067,19.1017490200354,-1.76117557468897));
#44820=CARTESIAN_POINT('Ctrl Pts',(-21.2938616787506,19.1843882419918,-1.76530286759568));
#44821=CARTESIAN_POINT('Ctrl Pts',(-21.293959303024,19.19377900214,-1.76577187513024));
#44822=CARTESIAN_POINT('Ctrl Pts',(-21.2940052315681,19.2031683255366,-1.76624088266481));
#44823=CARTESIAN_POINT('Ctrl Pts',(-21.2939995273705,19.2125555907563,-1.76670989019937));
#44824=CARTESIAN_POINT('Origin',(-18.734,19.211,1.76670989022852));
#44825=CARTESIAN_POINT('',(-17.1769962363369,21.2378222944355,-0.450077502023298));
#44826=CARTESIAN_POINT('',(-17.1722616682727,21.2439679654049,-0.516748662007315));
#44827=CARTESIAN_POINT('',(-17.1744642439897,21.2411350264762,1.76670989022852));
#44828=CARTESIAN_POINT('',(-21.2914665409842,19.2078565222202,-0.166709890228504));
#44829=CARTESIAN_POINT('Ctrl Pts',(-21.2914665409842,19.2078565222202,-0.166709890228504));
#44830=CARTESIAN_POINT('Ctrl Pts',(-21.286948837742,19.7963214614176,-0.195923797939959));
#44831=CARTESIAN_POINT('Ctrl Pts',(-20.7940989485341,21.2477394666147,-0.267529641211891));
#44832=CARTESIAN_POINT('Ctrl Pts',(-18.7954430158883,22.0506149083018,-0.361985511810154));
#44833=CARTESIAN_POINT('Ctrl Pts',(-17.5432452930182,21.517847446733,-0.427227474696966));
#44834=CARTESIAN_POINT('Ctrl Pts',(-17.1769962363369,21.2378222944355,-0.450077502023298));
#44835=CARTESIAN_POINT('',(-19.3957372685685,16.7380050975816,0.));
#44836=CARTESIAN_POINT('Ctrl Pts',(-19.3957372685684,16.7380050975816,1.38777878078145E-15));
#44837=CARTESIAN_POINT('Ctrl Pts',(-20.2191097516036,16.9583275322964,-0.0423919355604767));
#44838=CARTESIAN_POINT('Ctrl Pts',(-21.1334433095435,17.8262083452195,-0.0979618989699786));
#44839=CARTESIAN_POINT('Ctrl Pts',(-21.2935044203301,18.9424073589822,-0.153531862379481));
#44840=CARTESIAN_POINT('Ctrl Pts',(-21.2914665409842,19.2078565222202,-0.166709890228504));
#44841=CARTESIAN_POINT('',(-18.0722320621911,16.7380133044256,-1.80302994756687E-11));
#44842=CARTESIAN_POINT('Origin',(-18.734,19.211,0.));
#44843=CARTESIAN_POINT('',(-21.2939992552734,19.212952690406,-0.233290109771496));
#44844=CARTESIAN_POINT('Ctrl Pts',(-18.0722320621911,16.7380133044256,-1.80300219199125E-11));
#44845=CARTESIAN_POINT('Ctrl Pts',(-18.1529464922157,16.7164142307207,-0.00418158398862037));
#44846=CARTESIAN_POINT('Ctrl Pts',(-18.2348706569439,16.6987304519573,-0.00836316795921058));
#44847=CARTESIAN_POINT('Ctrl Pts',(-18.3175895998167,16.6850937510234,-0.012544751929801));
#44848=CARTESIAN_POINT('Ctrl Pts',(-18.400190747281,16.6714764693507,-0.0167203811411207));
#44849=CARTESIAN_POINT('Ctrl Pts',(-18.4835839741038,16.6618948926126,-0.0208960103524402));
#44850=CARTESIAN_POINT('Ctrl Pts',(-18.5673406239762,16.656430632693,-0.02507163956376));
#44851=CARTESIAN_POINT('Ctrl Pts',(-18.6514938546105,16.6509404999577,-0.0292670400316576));
#44852=CARTESIAN_POINT('Ctrl Pts',(-18.7360135046785,16.6496069028829,-0.0334624404995552));
#44853=CARTESIAN_POINT('Ctrl Pts',(-18.8204558534901,16.6524603021651,-0.0376578409674528));
#44854=CARTESIAN_POINT('Ctrl Pts',(-18.9043486080215,16.6552951300557,-0.0418259356091481));
#44855=CARTESIAN_POINT('Ctrl Pts',(-18.9881645984016,16.6622626001438,-0.0459940302508442));
#44856=CARTESIAN_POINT('Ctrl Pts',(-19.0714668099551,16.6733404183818,-0.0501621248925395));
#44857=CARTESIAN_POINT('Ctrl Pts',(-19.1547409379247,16.684414501967,-0.0543288143490282));
#44858=CARTESIAN_POINT('Ctrl Pts',(-19.2375011746968,16.6995961209329,-0.0584955038055169));
#44859=CARTESIAN_POINT('Ctrl Pts',(-19.3193159599542,16.7188111574315,-0.0626621932620057));
#44860=CARTESIAN_POINT('Ctrl Pts',(-19.4011278018881,16.7380255026606,-0.0668287328199814));
#44861=CARTESIAN_POINT('Ctrl Pts',(-19.481993811599,16.7612728705988,-0.0709952723779566));
#44862=CARTESIAN_POINT('Ctrl Pts',(-19.5614943032478,16.7884283956728,-0.0751618119359323));
#44863=CARTESIAN_POINT('Ctrl Pts',(-19.6419503629735,16.8159103206512,-0.0793784318407133));
#44864=CARTESIAN_POINT('Ctrl Pts',(-19.721007396075,16.8473948424126,-0.0835950517454946));
#44865=CARTESIAN_POINT('Ctrl Pts',(-19.7982496311477,16.8827017539409,-0.0878116716502757));
#44866=CARTESIAN_POINT('Ctrl Pts',(-19.8746816906651,16.9176383396154,-0.0919840644250511));
#44867=CARTESIAN_POINT('Ctrl Pts',(-19.9493364580842,16.9563172372311,-0.0961564571998266));
#44868=CARTESIAN_POINT('Ctrl Pts',(-20.0218360729121,16.9985176273456,-0.100328849974602));
#44869=CARTESIAN_POINT('Ctrl Pts',(-20.0954884255321,17.0413890001219,-0.104567583444386));
#44870=CARTESIAN_POINT('Ctrl Pts',(-20.1669160788343,17.0878945550855,-0.10880631691417));
#44871=CARTESIAN_POINT('Ctrl Pts',(-20.2357552271545,17.1377582780307,-0.113045050383954));
#44872=CARTESIAN_POINT('Ctrl Pts',(-20.3045943754748,17.187622000976,-0.117283783853738));
#44873=CARTESIAN_POINT('Ctrl Pts',(-20.370844676157,17.2408435335627,-0.121522517323522));
#44874=CARTESIAN_POINT('Ctrl Pts',(-20.4341804449292,17.2971069897509,-0.125761250793306));
#44875=CARTESIAN_POINT('Ctrl Pts',(-20.4958618563844,17.3519008204458,-0.129889266735435));
#44876=CARTESIAN_POINT('Ctrl Pts',(-20.5550187589506,17.4097927026216,-0.134017282677563));
#44877=CARTESIAN_POINT('Ctrl Pts',(-20.611317450137,17.4705175406195,-0.138145298619692));
#44878=CARTESIAN_POINT('Ctrl Pts',(-20.6675250696014,17.5311441469278,-0.142266636866263));
#44879=CARTESIAN_POINT('Ctrl Pts',(-20.7208833454928,17.5945942591679,-0.146387975112834));
#44880=CARTESIAN_POINT('Ctrl Pts',(-20.7710927993391,17.6605636333984,-0.150509313359405));
#44881=CARTESIAN_POINT('Ctrl Pts',(-20.8212566260777,17.7264730589238,-0.154626906400053));
#44882=CARTESIAN_POINT('Ctrl Pts',(-20.8682770216554,17.7948968304612,-0.158744499440701));
#44883=CARTESIAN_POINT('Ctrl Pts',(-20.9118931634006,17.8654958681547,-0.162862092481349));
#44884=CARTESIAN_POINT('Ctrl Pts',(-20.9554835923167,17.9360532859129,-0.166977258095768));
#44885=CARTESIAN_POINT('Ctrl Pts',(-20.9956735017905,18.0087830229833,-0.171092423710186));
#44886=CARTESIAN_POINT('Ctrl Pts',(-21.0322449058945,18.0833163774666,-0.175207589324605));
#44887=CARTESIAN_POINT('Ctrl Pts',(-21.0688064212004,18.1578295783544,-0.179321642210581));
#44888=CARTESIAN_POINT('Ctrl Pts',(-21.1017511664475,18.2341450028519,-0.183435695096556));
#44889=CARTESIAN_POINT('Ctrl Pts',(-21.1309074513388,18.3118700484822,-0.187549747982531));
#44890=CARTESIAN_POINT('Ctrl Pts',(-21.1600799709319,18.3896383727037,-0.19166609164121));
#44891=CARTESIAN_POINT('Ctrl Pts',(-21.1854596457913,18.4688174432781,-0.195782435299889));
#44892=CARTESIAN_POINT('Ctrl Pts',(-21.2069235819087,18.5489962552674,-0.199898778958568));
#44893=CARTESIAN_POINT('Ctrl Pts',(-21.228393434594,18.6291971686732,-0.204016257293894));
#44894=CARTESIAN_POINT('Ctrl Pts',(-21.2459452949941,18.710397909727,-0.208133735629219));
#44895=CARTESIAN_POINT('Ctrl Pts',(-21.259507205158,18.7921762223861,-0.212251213964544));
#44896=CARTESIAN_POINT('Ctrl Pts',(-21.2730871889122,18.8740635187863,-0.216374179551669));
#44897=CARTESIAN_POINT('Ctrl Pts',(-21.2826665466436,18.9565294532014,-0.220497145138794));
#44898=CARTESIAN_POINT('Ctrl Pts',(-21.2882251802136,19.0391461994527,-0.224620110725918));
#44899=CARTESIAN_POINT('Ctrl Pts',(-21.2921215137894,19.0970565470744,-0.227510110407777));
#44900=CARTESIAN_POINT('Ctrl Pts',(-21.2940434286409,19.1550409048321,-0.230400110089637));
#44901=CARTESIAN_POINT('Ctrl Pts',(-21.2939992552734,19.212952690406,-0.233290109771496));
#44902=CARTESIAN_POINT('Ctrl Pts',(-21.2960081472498,19.2129542227284,-0.233290109771496));
#44903=CARTESIAN_POINT('Ctrl Pts',(-21.2971424692952,19.3442911272882,-0.239839092339242));
#44904=CARTESIAN_POINT('Ctrl Pts',(-21.2281784359338,20.3246261525587,-0.288780010467465));
#44905=CARTESIAN_POINT('Ctrl Pts',(-19.9618263685217,21.9781789381743,-0.380112864156167));
#44906=CARTESIAN_POINT('Ctrl Pts',(-17.9636855616863,21.8141356871712,-0.468050065667029));
#44907=CARTESIAN_POINT('Ctrl Pts',(-17.2221125833706,21.2827383699607,-0.513595331617412));
#44908=CARTESIAN_POINT('Ctrl Pts',(-17.1722616682727,21.2439679654049,-0.516748662007315));
#44909=CARTESIAN_POINT('Origin',(18.734,19.211,1.76670989022852));
#44910=CARTESIAN_POINT('',(20.2955779010576,21.2437559712559,-21.2501821977678));
#44911=CARTESIAN_POINT('',(20.2916907287181,21.2386977908337,-21.3166133948081));
#44912=CARTESIAN_POINT('',(20.2935358855687,21.2411349269503,1.76670989022852));
#44913=CARTESIAN_POINT('',(16.1765333526442,19.2141444406009,-21.8332901097715));
#44914=CARTESIAN_POINT('Ctrl Pts',(20.291690728718,21.2386977908338,-21.3166133948081));
#44915=CARTESIAN_POINT('Ctrl Pts',(20.5461545344932,21.0458241145069,-21.3324492520697));
#44916=CARTESIAN_POINT('Ctrl Pts',(21.351877546268,20.1710072872175,-21.3906770448917));
#44917=CARTESIAN_POINT('Ctrl Pts',(21.4520480990298,17.8786570465205,-21.4912967732743));
#44918=CARTESIAN_POINT('Ctrl Pts',(19.0860574232626,16.2052798622314,-21.6184725799557));
#44919=CARTESIAN_POINT('Ctrl Pts',(16.6739013896572,17.1742593445012,-21.7324703587881));
#44920=CARTESIAN_POINT('Ctrl Pts',(16.1810511499193,18.6256790739174,-21.80407620206));
#44921=CARTESIAN_POINT('Ctrl Pts',(16.1765333526442,19.2141444406009,-21.8332901097715));
#44922=CARTESIAN_POINT('',(18.0722627314313,21.6839949024184,-22.));
#44923=CARTESIAN_POINT('Ctrl Pts',(16.1765333526442,19.2141444406009,-21.8332901097715));
#44924=CARTESIAN_POINT('Ctrl Pts',(16.1744954308812,19.4795937966726,-21.8464681376205));
#44925=CARTESIAN_POINT('Ctrl Pts',(16.3345564048251,20.5957933867983,-21.90203810103));
#44926=CARTESIAN_POINT('Ctrl Pts',(17.2488902483962,21.4636724677035,-21.9576080644395));
#44927=CARTESIAN_POINT('Ctrl Pts',(18.0722627314313,21.6839949024184,-22.));
#44928=CARTESIAN_POINT('',(19.3957680159044,21.6839866746762,-21.9999999999818));
#44929=CARTESIAN_POINT('Origin',(18.734,19.211,-22.));
#44930=CARTESIAN_POINT('',(16.1740007447408,19.2090472910618,-21.7667098902285));
#44931=CARTESIAN_POINT('Ctrl Pts',(16.1740007447408,19.2090472910617,-21.7667098902285));
#44932=CARTESIAN_POINT('Ctrl Pts',(16.1739377131957,19.291681576866,-21.770833628557));
#44933=CARTESIAN_POINT('Ctrl Pts',(16.1778799213038,19.3744638154111,-21.7749573668856));
#44934=CARTESIAN_POINT('Ctrl Pts',(16.1858438026722,19.4569674653686,-21.7790811052141));
#44935=CARTESIAN_POINT('Ctrl Pts',(16.1937978799175,19.539369547271,-21.7831997669178));
#44936=CARTESIAN_POINT('Ctrl Pts',(16.2057637505312,19.6214932533812,-21.7873184286214));
#44937=CARTESIAN_POINT('Ctrl Pts',(16.2217058123253,19.7029125070335,-21.7914370903251));
#44938=CARTESIAN_POINT('Ctrl Pts',(16.237637182478,19.7842771563645,-21.795552989823));
#44939=CARTESIAN_POINT('Ctrl Pts',(16.257539363199,19.864937827131,-21.799668889321));
#44940=CARTESIAN_POINT('Ctrl Pts',(16.2813251278132,19.9444752697558,-21.803784788819));
#44941=CARTESIAN_POINT('Ctrl Pts',(16.3051025310591,20.0239847527225,-21.807899241462));
#44942=CARTESIAN_POINT('Ctrl Pts',(16.3327606729939,20.1023713378542,-21.812013694105));
#44943=CARTESIAN_POINT('Ctrl Pts',(16.3641619718452,20.1792291672488,-21.816128146748));
#44944=CARTESIAN_POINT('Ctrl Pts',(16.3955622525032,20.2560845045131,-21.820242465979));
#44945=CARTESIAN_POINT('Ctrl Pts',(16.4307052681111,20.331410746752,-21.8243567852101));
#44946=CARTESIAN_POINT('Ctrl Pts',(16.4694052055202,20.4048217692834,-21.8284711044412));
#44947=CARTESIAN_POINT('Ctrl Pts',(16.5081407935446,20.4783004184906,-21.8325892138079));
#44948=CARTESIAN_POINT('Ctrl Pts',(16.5504396244287,20.5498599054295,-21.8367073231746));
#44949=CARTESIAN_POINT('Ctrl Pts',(16.596070140308,20.6191391674964,-21.8408254325413));
#44950=CARTESIAN_POINT('Ctrl Pts',(16.6417225473624,20.6884516661905,-21.8449455175651));
#44951=CARTESIAN_POINT('Ctrl Pts',(16.6907095403228,20.7554813807654,-21.849065602589));
#44952=CARTESIAN_POINT('Ctrl Pts',(16.7427579777409,20.819898756538,-21.8531856876128));
#44953=CARTESIAN_POINT('Ctrl Pts',(16.7948924451882,20.88442260676,-21.8573125826592));
#44954=CARTESIAN_POINT('Ctrl Pts',(16.8500981442698,20.9463251442536,-21.8614394777056));
#44955=CARTESIAN_POINT('Ctrl Pts',(16.9080639888335,21.0053125934813,-21.865566372752));
#44956=CARTESIAN_POINT('Ctrl Pts',(16.9486676888643,21.0466319033619,-21.8684571649036));
#44957=CARTESIAN_POINT('Ctrl Pts',(16.990624926523,21.0865216582628,-21.8713479570551));
#44958=CARTESIAN_POINT('Ctrl Pts',(17.0338195605382,21.124893015106,-21.8742387492067));
#44959=CARTESIAN_POINT('Ctrl Pts',(17.096294549636,21.1803918092294,-21.8784198752255));
#44960=CARTESIAN_POINT('Ctrl Pts',(17.1616053008015,21.2329308852276,-21.8826010012442));
#44961=CARTESIAN_POINT('Ctrl Pts',(17.2294394909469,21.2822068159887,-21.886782127263));
#44962=CARTESIAN_POINT('Ctrl Pts',(17.2971786580471,21.3314137203636,-21.8909573963043));
#44963=CARTESIAN_POINT('Ctrl Pts',(17.3674338732044,21.377366290339,-21.8951326653455));
#44964=CARTESIAN_POINT('Ctrl Pts',(17.4398581404809,21.4197998658639,-21.8993079343868));
#44965=CARTESIAN_POINT('Ctrl Pts',(17.5126333816213,21.462439077932,-21.9035034371199));
#44966=CARTESIAN_POINT('Ctrl Pts',(17.5875984040009,21.5015247814357,-21.907698939853));
#44967=CARTESIAN_POINT('Ctrl Pts',(17.6643697795486,21.5368312904201,-21.9118944425862));
#44968=CARTESIAN_POINT('Ctrl Pts',(17.7406374344996,21.5719061425448,-21.916062417336));
#44969=CARTESIAN_POINT('Ctrl Pts',(17.8186873858889,21.603251049355,-21.9202303920859));
#44970=CARTESIAN_POINT('Ctrl Pts',(17.8981187211547,21.6306905768457,-21.9243983668358));
#44971=CARTESIAN_POINT('Ctrl Pts',(17.9775250004187,21.6581214487492,-21.9285650268302));
#44972=CARTESIAN_POINT('Ctrl Pts',(18.0583113629463,21.681649237629,-21.9327316868246));
#44973=CARTESIAN_POINT('Ctrl Pts',(18.1400586239765,21.7011473132823,-21.936898346819));
#44974=CARTESIAN_POINT('Ctrl Pts',(18.2218047170262,21.720645110353,-21.9410649472815));
#44975=CARTESIAN_POINT('Ctrl Pts',(18.3045112328003,21.7361132028771,-21.9452315477439));
#44976=CARTESIAN_POINT('Ctrl Pts',(18.3877469394689,21.7474756687327,-21.9493981482063));
#44977=CARTESIAN_POINT('Ctrl Pts',(18.471985895769,21.7589750877077,-21.9536149691876));
#44978=CARTESIAN_POINT('Ctrl Pts',(18.5567664092282,21.7662691624329,-21.9578317901689));
#44979=CARTESIAN_POINT('Ctrl Pts',(18.6416360132955,21.7693332257468,-21.9620486111502));
#44980=CARTESIAN_POINT('Ctrl Pts',(18.7256171152011,21.7723652112997,-21.9662212861195));
#44981=CARTESIAN_POINT('Ctrl Pts',(18.8096849858173,21.7712554086671,-21.9703939610888));
#44982=CARTESIAN_POINT('Ctrl Pts',(18.8934029358148,21.766032427202,-21.9745666360581));
#44983=CARTESIAN_POINT('Ctrl Pts',(18.9784494629181,21.7607265586906,-21.9788055300454));
#44984=CARTESIAN_POINT('Ctrl Pts',(19.0631343741421,21.7511758815698,-21.9830444240327));
#44985=CARTESIAN_POINT('Ctrl Pts',(19.1470089679579,21.7374646430113,-21.98728331802));
#44986=CARTESIAN_POINT('Ctrl Pts',(19.2308835617738,21.7237534044529,-21.9915222120073));
#44987=CARTESIAN_POINT('Ctrl Pts',(19.3139473718607,21.7058817725444,-21.9957611059945));
#44988=CARTESIAN_POINT('Ctrl Pts',(19.3957680159044,21.6839866746762,-21.9999999999818));
#44989=CARTESIAN_POINT('Ctrl Pts',(20.2955779010576,21.2437559712559,-21.2501821977678));
#44990=CARTESIAN_POINT('Ctrl Pts',(20.9031380122802,20.7701939876851,-21.2886333060055));
#44991=CARTESIAN_POINT('Ctrl Pts',(21.7186680886982,19.1595846939594,-21.3694763498038));
#44992=CARTESIAN_POINT('Ctrl Pts',(20.3959082140047,16.6810622569708,-21.4927113291624));
#44993=CARTESIAN_POINT('Ctrl Pts',(17.5061735829933,16.443821090153,-21.6198871358438));
#44994=CARTESIAN_POINT('Ctrl Pts',(16.2398215703271,18.0973737800013,-21.7112199895325));
#44995=CARTESIAN_POINT('Ctrl Pts',(16.1708575106781,19.0777088474958,-21.7601609076608));
#44996=CARTESIAN_POINT('Ctrl Pts',(16.1719918287103,19.2090457587065,-21.7667098902285));
#44997=CARTESIAN_POINT('Origin',(18.734,19.211,1.76670989022852));
#44998=CARTESIAN_POINT('',(20.294072606836,21.2418453397989,-20.4499991791617));
#44999=CARTESIAN_POINT('',(20.2935358855687,21.2411349269503,-20.5167505016347));
#45000=CARTESIAN_POINT('',(20.2935358855687,21.2411349269503,1.76670989022852));
#45001=CARTESIAN_POINT('',(16.1740711622283,19.2096583021525,-21.0332900817674));
#45002=CARTESIAN_POINT('Ctrl Pts',(20.2935358855687,21.2411349269503,-20.5167505016347));
#45003=CARTESIAN_POINT('Ctrl Pts',(20.3601729811252,21.1899447619761,-20.5209209409253));
#45004=CARTESIAN_POINT('Ctrl Pts',(20.424326855727,21.135439617875,-20.5250913802159));
#45005=CARTESIAN_POINT('Ctrl Pts',(20.4856569022985,21.0778953094991,-20.5292618195065));
#45006=CARTESIAN_POINT('Ctrl Pts',(20.5469737333947,21.020363400843,-20.5334313601456));
#45007=CARTESIAN_POINT('Ctrl Pts',(20.6054676099457,20.9597939435863,-20.5376009007847));
#45008=CARTESIAN_POINT('Ctrl Pts',(20.6608329431096,20.8965013525203,-20.5417704414238));
#45009=CARTESIAN_POINT('Ctrl Pts',(20.7162029534294,20.8332034146189,-20.5459403342977));
#45010=CARTESIAN_POINT('Ctrl Pts',(20.768443593682,20.7671822332372,-20.5501102271715));
#45011=CARTESIAN_POINT('Ctrl Pts',(20.8172888253184,20.6987861641726,-20.5542801200453));
#45012=CARTESIAN_POINT('Ctrl Pts',(20.8661854255174,20.6303181657171,-20.5584543982275));
#45013=CARTESIAN_POINT('Ctrl Pts',(20.9116792192141,20.5594706676898,-20.5626286764097));
#45014=CARTESIAN_POINT('Ctrl Pts',(20.9535471859618,20.4866215305838,-20.5668029545919));
#45015=CARTESIAN_POINT('Ctrl Pts',(20.9954381169732,20.4137324362761,-20.5709795223342));
#45016=CARTESIAN_POINT('Ctrl Pts',(21.0336990517046,20.3388399266131,-20.5751560900764));
#45017=CARTESIAN_POINT('Ctrl Pts',(21.0681538129048,20.262344842429,-20.5793326578187));
#45018=CARTESIAN_POINT('Ctrl Pts',(21.102668195464,20.1857173892858,-20.5835164527956));
#45019=CARTESIAN_POINT('Ctrl Pts',(21.1333630817951,20.1074822515155,-20.5877002477726));
#45020=CARTESIAN_POINT('Ctrl Pts',(21.1601112326058,20.0280583131111,-20.5918840427495));
#45021=CARTESIAN_POINT('Ctrl Pts',(21.1796790940316,19.9699549835918,-20.5949447373344));
#45022=CARTESIAN_POINT('Ctrl Pts',(21.1971357839931,19.9112157932946,-20.5980054319194));
#45023=CARTESIAN_POINT('Ctrl Pts',(21.2124488472496,19.8520080432935,-20.6010661265043));
#45024=CARTESIAN_POINT('Ctrl Pts',(21.2333845649191,19.7710603767749,-20.6052506476957));
#45025=CARTESIAN_POINT('Ctrl Pts',(21.2503893834586,19.6889352855203,-20.6094351688871));
#45026=CARTESIAN_POINT('Ctrl Pts',(21.2633350895848,19.60604936982,-20.6136196900785));
#45027=CARTESIAN_POINT('Ctrl Pts',(21.2762623681897,19.5232814377936,-20.6177982548275));
#45028=CARTESIAN_POINT('Ctrl Pts',(21.2851419407631,19.4397552831428,-20.6219768195765));
#45029=CARTESIAN_POINT('Ctrl Pts',(21.2898958841357,19.3559007572729,-20.6261553843254));
#45030=CARTESIAN_POINT('Ctrl Pts',(21.2947352019949,19.2705403158833,-20.630408990528));
#45031=CARTESIAN_POINT('Ctrl Pts',(21.2952991221744,19.1848400591974,-20.6346625967305));
#45032=CARTESIAN_POINT('Ctrl Pts',(21.291560298618,19.099262276142,-20.638916202933));
#45033=CARTESIAN_POINT('Ctrl Pts',(21.2878940830536,19.0153464145152,-20.6430872040592));
#45034=CARTESIAN_POINT('Ctrl Pts',(21.2800907693894,18.9315487929963,-20.6472582051854));
#45035=CARTESIAN_POINT('Ctrl Pts',(21.2681770979566,18.848306691277,-20.6514292063116));
#45036=CARTESIAN_POINT('Ctrl Pts',(21.2562674231734,18.7650925145781,-20.6555988082025));
#45037=CARTESIAN_POINT('Ctrl Pts',(21.2402501942426,18.6824339426084,-20.6597684100934));
#45038=CARTESIAN_POINT('Ctrl Pts',(21.2202039193129,18.6007622827183,-20.6639380119843));
#45039=CARTESIAN_POINT('Ctrl Pts',(21.200158355009,18.519093518029,-20.6681074660658));
#45040=CARTESIAN_POINT('Ctrl Pts',(21.1760841391767,18.4384120424547,-20.6722769201474));
#45041=CARTESIAN_POINT('Ctrl Pts',(21.1481104103814,18.359136791211,-20.6764463742289));
#45042=CARTESIAN_POINT('Ctrl Pts',(21.1191514849296,18.2770695735108,-20.6807626708086));
#45043=CARTESIAN_POINT('Ctrl Pts',(21.0860134223639,18.196509977735,-20.6850789673883));
#45044=CARTESIAN_POINT('Ctrl Pts',(21.0488942540618,18.1179013802444,-20.6893952639681));
#45045=CARTESIAN_POINT('Ctrl Pts',(21.0129862924118,18.0418577986349,-20.693570718838));
#45046=CARTESIAN_POINT('Ctrl Pts',(20.973353301174,17.9676402439562,-20.697746173708));
#45047=CARTESIAN_POINT('Ctrl Pts',(20.93022101813,17.8956242971971,-20.7019216285779));
#45048=CARTESIAN_POINT('Ctrl Pts',(20.8849064011798,17.8199646100352,-20.7063083460125));
#45049=CARTESIAN_POINT('Ctrl Pts',(20.8357293767458,17.7467356778436,-20.7106950634472));
#45050=CARTESIAN_POINT('Ctrl Pts',(20.783001266459,17.6763359292505,-20.7150817808818));
#45051=CARTESIAN_POINT('Ctrl Pts',(20.7302731561721,17.6059361806573,-20.7194684983164));
#45052=CARTESIAN_POINT('Ctrl Pts',(20.6739943900424,17.5383660129748,-20.723855215751));
#45053=CARTESIAN_POINT('Ctrl Pts',(20.6145211534981,17.4739795075341,-20.7282419331856));
#45054=CARTESIAN_POINT('Ctrl Pts',(20.557786240175,17.412557546706,-20.7324266732114));
#45055=CARTESIAN_POINT('Ctrl Pts',(20.4979333333722,17.3538038540671,-20.7366114132371));
#45056=CARTESIAN_POINT('Ctrl Pts',(20.4352433666198,17.2980517499074,-20.7407961532628));
#45057=CARTESIAN_POINT('Ctrl Pts',(20.3726426389602,17.2423790088015,-20.7449749363161));
#45058=CARTESIAN_POINT('Ctrl Pts',(20.3072132139949,17.1896996722069,-20.7491537193694));
#45059=CARTESIAN_POINT('Ctrl Pts',(20.2392743867932,17.1403119451582,-20.7533325024227));
#45060=CARTESIAN_POINT('Ctrl Pts',(20.1701199701232,17.0900405525631,-20.7575860539829));
#45061=CARTESIAN_POINT('Ctrl Pts',(20.0983657943851,17.0431800747247,-20.7618396055431));
#45062=CARTESIAN_POINT('Ctrl Pts',(20.0243857326348,17.0000036949347,-20.7660931571032));
#45063=CARTESIAN_POINT('Ctrl Pts',(19.9518376849991,16.9576630698576,-20.7702643736974));
#45064=CARTESIAN_POINT('Ctrl Pts',(19.877149571062,16.9188654316441,-20.7744355902916));
#45065=CARTESIAN_POINT('Ctrl Pts',(19.8007035800232,16.8838250017745,-20.7786068068857));
#45066=CARTESIAN_POINT('Ctrl Pts',(19.7242832605526,16.8487963389417,-20.7827766227305));
#45067=CARTESIAN_POINT('Ctrl Pts',(19.6461066541874,16.8175225701701,-20.7869464385753));
#45068=CARTESIAN_POINT('Ctrl Pts',(19.5665789492871,16.7901711557394,-20.7911162544201));
#45069=CARTESIAN_POINT('Ctrl Pts',(19.487054097481,16.7628207225537,-20.7952859206708));
#45070=CARTESIAN_POINT('Ctrl Pts',(19.4061786787909,16.739392512731,-20.7994555869215));
#45071=CARTESIAN_POINT('Ctrl Pts',(19.3243748845357,16.7200047178468,-20.8036252531722));
#45072=CARTESIAN_POINT('Ctrl Pts',(19.2396994039173,16.699936322916,-20.8079412937301));
#45073=CARTESIAN_POINT('Ctrl Pts',(19.1540296670697,16.6841974189308,-20.812257334288));
#45074=CARTESIAN_POINT('Ctrl Pts',(19.0678455536436,16.6728614800779,-20.816573374846));
#45075=CARTESIAN_POINT('Ctrl Pts',(18.9844645957683,16.6618942449066,-20.8207490353203));
#45076=CARTESIAN_POINT('Ctrl Pts',(18.9006026820952,16.655047941956,-20.8249246957946));
#45077=CARTESIAN_POINT('Ctrl Pts',(18.8166978402032,16.6523360777105,-20.8291003562689));
#45078=CARTESIAN_POINT('Ctrl Pts',(18.7285618465719,16.6494874596275,-20.8334865868686));
#45079=CARTESIAN_POINT('Ctrl Pts',(18.6403790648446,16.6512012136138,-20.8378728174683));
#45080=CARTESIAN_POINT('Ctrl Pts',(18.5526528284857,16.6574312808574,-20.842259048068));
#45081=CARTESIAN_POINT('Ctrl Pts',(18.4649265921268,16.6636613481009,-20.8466452786677));
#45082=CARTESIAN_POINT('Ctrl Pts',(18.377657467477,16.674407582305,-20.8510315092674));
#45083=CARTESIAN_POINT('Ctrl Pts',(18.291335798662,16.6895622345864,-20.8554177398671));
#45084=CARTESIAN_POINT('Ctrl Pts',(18.2089776381982,16.7040210524186,-20.8596025742027));
#45085=CARTESIAN_POINT('Ctrl Pts',(18.1271754855616,16.7225461173931,-20.8637874085383));
#45086=CARTESIAN_POINT('Ctrl Pts',(18.0463616920216,16.7450815996062,-20.8679722428739));
#45087=CARTESIAN_POINT('Ctrl Pts',(17.9656628851168,16.7675850170052,-20.8721511227802));
#45088=CARTESIAN_POINT('Ctrl Pts',(17.8859500832462,16.7940873946837,-20.8763300026865));
#45089=CARTESIAN_POINT('Ctrl Pts',(17.8076468720086,16.8244816400747,-20.8805088825927));
#45090=CARTESIAN_POINT('Ctrl Pts',(17.7279449225119,16.8554188209751,-20.8847624102576));
#45091=CARTESIAN_POINT('Ctrl Pts',(17.6497038935225,16.8903881967178,-20.8890159379224));
#45092=CARTESIAN_POINT('Ctrl Pts',(17.5733558329037,16.9292232542632,-20.8932694655872));
#45093=CARTESIAN_POINT('Ctrl Pts',(17.4984833659798,16.9673077391602,-20.8974407845024));
#45094=CARTESIAN_POINT('Ctrl Pts',(17.4254317755317,17.0091095912714,-20.9016121034175));
#45095=CARTESIAN_POINT('Ctrl Pts',(17.3545880686222,17.0544233786919,-20.9057834223326));
#45096=CARTESIAN_POINT('Ctrl Pts',(17.2837681207939,17.0997219690822,-20.9099533422992));
#45097=CARTESIAN_POINT('Ctrl Pts',(17.2151549730963,17.1485299079791,-20.9141232622657));
#45098=CARTESIAN_POINT('Ctrl Pts',(17.1491087606961,17.2005971151091,-20.9182931822323));
#45099=CARTESIAN_POINT('Ctrl Pts',(17.0830648915161,17.2526624749729,-20.9224629542563));
#45100=CARTESIAN_POINT('Ctrl Pts',(17.0195881372622,17.3079865877152,-20.9266327262804));
#45101=CARTESIAN_POINT('Ctrl Pts',(16.9590064076373,17.3662784093334,-20.9308024983044));
#45102=CARTESIAN_POINT('Ctrl Pts',(16.8963013152165,17.426613333486,-20.9351184189914));
#45103=CARTESIAN_POINT('Ctrl Pts',(16.8366983378611,17.4901275014,-20.9394343396785));
#45104=CARTESIAN_POINT('Ctrl Pts',(16.7805189594486,17.5564572159638,-20.9437502603655));
#45105=CARTESIAN_POINT('Ctrl Pts',(16.7261639013718,17.6206329969926,-20.947926029593));
#45106=CARTESIAN_POINT('Ctrl Pts',(16.675013743749,17.6874438611075,-20.9521017988205));
#45107=CARTESIAN_POINT('Ctrl Pts',(16.6273169449433,17.7565287883437,-20.9562775680481));
#45108=CARTESIAN_POINT('Ctrl Pts',(16.5772188726476,17.8290917645997,-20.9606635644648));
#45109=CARTESIAN_POINT('Ctrl Pts',(16.5309313071793,17.9041632904916,-20.9650495608815));
#45110=CARTESIAN_POINT('Ctrl Pts',(16.4886879176911,17.9812952984404,-20.9694355572983));
#45111=CARTESIAN_POINT('Ctrl Pts',(16.446444528203,18.0584273063893,-20.973821553715));
#45112=CARTESIAN_POINT('Ctrl Pts',(16.4082454981438,18.137619241256,-20.9782075501317));
#45113=CARTESIAN_POINT('Ctrl Pts',(16.3742656129549,18.2184005729416,-20.9825935465485));
#45114=CARTESIAN_POINT('Ctrl Pts',(16.3382155097944,18.3041034917275,-20.9872467589536));
#45115=CARTESIAN_POINT('Ctrl Pts',(16.306798874077,18.3918657738651,-20.9918999713587));
#45116=CARTESIAN_POINT('Ctrl Pts',(16.2802296051744,18.4811980751755,-20.9965531837637));
#45117=CARTESIAN_POINT('Ctrl Pts',(16.2537435497692,18.5702505926029,-21.001191822562));
#45118=CARTESIAN_POINT('Ctrl Pts',(16.2320746945689,18.6608630689237,-21.0058304613603));
#45119=CARTESIAN_POINT('Ctrl Pts',(16.2153886002422,18.752527953949,-21.0104691001586));
#45120=CARTESIAN_POINT('Ctrl Pts',(16.1987928060345,18.8436967762135,-21.0150826360402));
#45121=CARTESIAN_POINT('Ctrl Pts',(16.1871261070645,18.9359063886952,-21.0196961719218));
#45122=CARTESIAN_POINT('Ctrl Pts',(16.1805035110245,19.0286385984106,-21.0243097078035));
#45123=CARTESIAN_POINT('Ctrl Pts',(16.1762064897689,19.0888071899736,-21.0273031655996));
#45124=CARTESIAN_POINT('Ctrl Pts',(16.1740320413884,19.1491954186321,-21.0302966233957));
#45125=CARTESIAN_POINT('Ctrl Pts',(16.174000351618,19.2096582534287,-21.0332900811918));
#45126=CARTESIAN_POINT('Ctrl Pts',(16.1775161339837,19.2096606725892,-21.0332901097715));
#45127=CARTESIAN_POINT('Ctrl Pts',(16.1799699186122,19.7238724897518,-21.0587831909243));
#45128=CARTESIAN_POINT('Ctrl Pts',(16.5801691862074,21.0966582496844,-21.1266682076376));
#45129=CARTESIAN_POINT('Ctrl Pts',(18.4990491868353,22.0730068113866,-21.2211093026498));
#45130=CARTESIAN_POINT('Ctrl Pts',(19.864965440735,21.5621389766016,-21.2900573165092));
#45131=CARTESIAN_POINT('Ctrl Pts',(20.291690728718,21.2386977908338,-21.3166133948081));
#45132=CARTESIAN_POINT('',(16.1715627854608,19.2128544306465,-20.9667098902285));
#45133=CARTESIAN_POINT('Ctrl Pts',(16.1715627854608,19.2128544306465,-20.9667098902285));
#45134=CARTESIAN_POINT('Ctrl Pts',(16.1706209869532,19.3284704702211,-20.9724759609646));
#45135=CARTESIAN_POINT('Ctrl Pts',(16.2303035804914,20.2931122226394,-21.0206339672611));
#45136=CARTESIAN_POINT('Ctrl Pts',(17.4553333859632,21.9547543997083,-21.1111839091181));
#45137=CARTESIAN_POINT('Ctrl Pts',(19.4740835948961,21.8268017090075,-21.1999086075618));
#45138=CARTESIAN_POINT('Ctrl Pts',(20.2333094880972,21.2922910093709,-21.246241370445));
#45139=CARTESIAN_POINT('Ctrl Pts',(20.2955779010576,21.2437559712559,-21.2501821977678));
#45140=CARTESIAN_POINT('Ctrl Pts',(20.2940726068359,21.241845339799,-20.4499991791617));
#45141=CARTESIAN_POINT('Ctrl Pts',(20.429454357434,21.1400081300327,-20.4584344113448));
#45142=CARTESIAN_POINT('Ctrl Pts',(21.1817798668074,20.4464549008743,-20.5092615790883));
#45143=CARTESIAN_POINT('Ctrl Pts',(21.642413960578,18.3717008291089,-20.6024806823923));
#45144=CARTESIAN_POINT('Ctrl Pts',(19.6025526335179,16.3111911491892,-20.7296564890738));
#45145=CARTESIAN_POINT('Ctrl Pts',(16.8944629772976,16.8838679918332,-20.8510662250192));
#45146=CARTESIAN_POINT('Ctrl Pts',(16.1775450542205,18.4784656881504,-20.9300840254041));
#45147=CARTESIAN_POINT('Ctrl Pts',(16.1715627854608,19.2128544306465,-20.9667098902285));
#45148=CARTESIAN_POINT('Origin',(18.734,19.211,1.76670989022852));
#45149=CARTESIAN_POINT('',(20.2935358855687,21.2411349269503,-19.6501081158318));
#45150=CARTESIAN_POINT('',(20.2935358855687,21.2411349269503,-19.7167245524671));
#45151=CARTESIAN_POINT('',(20.2935358855687,21.2411349269503,1.76670989022852));
#45152=CARTESIAN_POINT('',(16.1740004726297,19.2094444088938,-20.2332901098006));
#45153=CARTESIAN_POINT('Ctrl Pts',(20.2935358855687,21.2411349269503,-19.7167245524671));
#45154=CARTESIAN_POINT('Ctrl Pts',(20.3599060616565,21.1901498077021,-19.7209062209711));
#45155=CARTESIAN_POINT('Ctrl Pts',(20.423885153381,21.1358206778254,-19.7250878894751));
#45156=CARTESIAN_POINT('Ctrl Pts',(20.4851178678972,21.0784009244753,-19.7292695579791));
#45157=CARTESIAN_POINT('Ctrl Pts',(20.5462729398852,21.0210539788531,-19.7334459241653));
#45158=CARTESIAN_POINT('Ctrl Pts',(20.6046882194149,20.9606245074412,-19.7376222903514));
#45159=CARTESIAN_POINT('Ctrl Pts',(20.6600404272569,20.8974069119201,-19.7417986565376));
#45160=CARTESIAN_POINT('Ctrl Pts',(20.715340321286,20.8342490638527,-19.7459710756067));
#45161=CARTESIAN_POINT('Ctrl Pts',(20.7675825950387,20.7683086732424,-19.7501434946759));
#45162=CARTESIAN_POINT('Ctrl Pts',(20.8164808480404,20.6999168941029,-19.7543159137451));
#45163=CARTESIAN_POINT('Ctrl Pts',(20.8653546227575,20.6315593516349,-19.7584862441167));
#45164=CARTESIAN_POINT('Ctrl Pts',(20.9108874334552,20.5607532307721,-19.7626565744883));
#45165=CARTESIAN_POINT('Ctrl Pts',(20.9528339565094,20.4878617283954,-19.76682690486));
#45166=CARTESIAN_POINT('Ctrl Pts',(20.9947720643174,20.4149848493985,-19.7709963985864));
#45167=CARTESIAN_POINT('Ctrl Pts',(21.0331250845316,20.3400238186815,-19.7751658923128));
#45168=CARTESIAN_POINT('Ctrl Pts',(21.0676924581133,20.2633685243036,-19.7793353860393));
#45169=CARTESIAN_POINT('Ctrl Pts',(21.1022632661089,20.1867056139,-19.7835052940224));
#45170=CARTESIAN_POINT('Ctrl Pts',(21.1330474927277,20.1083485254935,-19.7876752020056));
#45171=CARTESIAN_POINT('Ctrl Pts',(21.1598923165065,20.0287080583649,-19.7918451099887));
#45172=CARTESIAN_POINT('Ctrl Pts',(21.1867656112298,19.948983126561,-19.7960194404714));
#45173=CARTESIAN_POINT('Ctrl Pts',(21.2096910141566,19.8679725352515,-19.800193770954));
#45174=CARTESIAN_POINT('Ctrl Pts',(21.2285654629023,19.7861027310794,-19.8043681014367));
#45175=CARTESIAN_POINT('Ctrl Pts',(21.2474505163374,19.7041869280093,-19.8085447772847));
#45176=CARTESIAN_POINT('Ctrl Pts',(21.2622800027704,19.6214114038201,-19.8127214531326));
#45177=CARTESIAN_POINT('Ctrl Pts',(21.2730023683084,19.5382109009864,-19.8168981289806));
#45178=CARTESIAN_POINT('Ctrl Pts',(21.2837431247208,19.4548676936352,-19.8210819686136));
#45179=CARTESIAN_POINT('Ctrl Pts',(21.2903626558656,19.3710985107369,-19.8252658082466));
#45180=CARTESIAN_POINT('Ctrl Pts',(21.2928614750997,19.2873410194495,-19.8294496478795));
#45181=CARTESIAN_POINT('Ctrl Pts',(21.2945659689719,19.230208383083,-19.8323035273916));
#45182=CARTESIAN_POINT('Ctrl Pts',(21.2943542420741,19.173081197621,-19.8351574069036));
#45183=CARTESIAN_POINT('Ctrl Pts',(21.2922402934572,19.1160968866051,-19.8380112864157));
#45184=CARTESIAN_POINT('Ctrl Pts',(21.2891406189063,19.0325410152651,-19.8421959187307));
#45185=CARTESIAN_POINT('Ctrl Pts',(21.2819372856915,18.9489816686976,-19.8463805510458));
#45186=CARTESIAN_POINT('Ctrl Pts',(21.2706266468752,18.8658547344046,-19.8505651833609));
#45187=CARTESIAN_POINT('Ctrl Pts',(21.2593321073605,18.7828461210669,-19.8547438593671));
#45188=CARTESIAN_POINT('Ctrl Pts',(21.2439419362161,18.70026914939,-19.8589225353733));
#45189=CARTESIAN_POINT('Ctrl Pts',(21.2245044655678,18.6185580138218,-19.8631012113796));
#45190=CARTESIAN_POINT('Ctrl Pts',(21.2047185799734,18.5353822133593,-19.8673547897845));
#45191=CARTESIAN_POINT('Ctrl Pts',(21.1807388847065,18.4531040774616,-19.8716083681894));
#45192=CARTESIAN_POINT('Ctrl Pts',(21.1526714444899,18.3721743663851,-19.8758619465942));
#45193=CARTESIAN_POINT('Ctrl Pts',(21.1251481633401,18.2928136846083,-19.8800330585099));
#45194=CARTESIAN_POINT('Ctrl Pts',(21.0936943831903,18.2147500635837,-19.8842041704256));
#45195=CARTESIAN_POINT('Ctrl Pts',(21.0584608475173,18.1383948683887,-19.8883752823413));
#45196=CARTESIAN_POINT('Ctrl Pts',(21.0232391347176,18.0620652947434,-19.8925449946096));
#45197=CARTESIAN_POINT('Ctrl Pts',(20.9842403778953,17.9874434257541,-19.8967147068778));
#45198=CARTESIAN_POINT('Ctrl Pts',(20.9416632153501,17.9149200921278,-19.9008844191461));
#45199=CARTESIAN_POINT('Ctrl Pts',(20.8990875677533,17.8423993389718,-19.9050539830508));
#45200=CARTESIAN_POINT('Ctrl Pts',(20.8529340012278,17.7719773690056,-19.9092235469555));
#45201=CARTESIAN_POINT('Ctrl Pts',(20.8034461281343,17.7040186720632,-19.9133931108602));
#45202=CARTESIAN_POINT('Ctrl Pts',(20.7522182683685,17.6336705568746,-19.9177092760466));
#45203=CARTESIAN_POINT('Ctrl Pts',(20.697417574011,17.5659625868841,-19.922025441233));
#45204=CARTESIAN_POINT('Ctrl Pts',(20.6393606094928,17.5012629009719,-19.9263416064194));
#45205=CARTESIAN_POINT('Ctrl Pts',(20.5831949030629,17.4386708658007,-19.9305171686242));
#45206=CARTESIAN_POINT('Ctrl Pts',(20.523982185993,17.3788944303194,-19.9346927308289));
#45207=CARTESIAN_POINT('Ctrl Pts',(20.4620462260796,17.3222289073231,-19.9388682930336));
#45208=CARTESIAN_POINT('Ctrl Pts',(20.3969819279172,17.2627012518396,-19.9432547597108));
#45209=CARTESIAN_POINT('Ctrl Pts',(20.3289124964447,17.206607414148,-19.9476412263881));
#45210=CARTESIAN_POINT('Ctrl Pts',(20.2582501417826,17.1542400467542,-19.9520276930653));
#45211=CARTESIAN_POINT('Ctrl Pts',(20.1875877871204,17.1018726793603,-19.9564141597426));
#45212=CARTESIAN_POINT('Ctrl Pts',(20.1143330347148,17.0532320398492,-19.9608006264198));
#45213=CARTESIAN_POINT('Ctrl Pts',(20.0389283877504,17.0085554711087,-19.965187093097));
#45214=CARTESIAN_POINT('Ctrl Pts',(19.9669932812562,16.9659345735974,-19.9693717283982));
#45215=CARTESIAN_POINT('Ctrl Pts',(19.8928340180633,16.9267623273783,-19.9735563636994));
#45216=CARTESIAN_POINT('Ctrl Pts',(19.8168151370682,16.8912777366814,-19.9777409990006));
#45217=CARTESIAN_POINT('Ctrl Pts',(19.7409044598177,16.8558436540364,-19.9819196779762));
#45218=CARTESIAN_POINT('Ctrl Pts',(19.6631398357153,16.8240869937955,-19.9860983569517));
#45219=CARTESIAN_POINT('Ctrl Pts',(19.5839125153273,16.796202137592,-19.9902770359273));
#45220=CARTESIAN_POINT('Ctrl Pts',(19.5032651236343,16.7678174729394,-19.9945306135878));
#45221=CARTESIAN_POINT('Ctrl Pts',(19.4211024978258,16.7434450253959,-19.9987841912482));
#45222=CARTESIAN_POINT('Ctrl Pts',(19.337861066102,16.7232395989874,-20.0030377689087));
#45223=CARTESIAN_POINT('Ctrl Pts',(19.2562334111056,16.7034258891344,-20.0072088837319));
#45224=CARTESIAN_POINT('Ctrl Pts',(19.1735688735385,16.6876191861435,-20.0113799985551));
#45225=CARTESIAN_POINT('Ctrl Pts',(19.0902949413653,16.6759154028401,-20.0155511133783));
#45226=CARTESIAN_POINT('Ctrl Pts',(19.0070489529371,16.6642155469066,-20.019720828525));
#45227=CARTESIAN_POINT('Ctrl Pts',(18.9231944312015,16.6566159403015,-20.0238905436717));
#45228=CARTESIAN_POINT('Ctrl Pts',(18.8391675225352,16.6531611090212,-20.0280602588184));
#45229=CARTESIAN_POINT('Ctrl Pts',(18.7551436043077,16.649706400695,-20.0322298255688));
#45230=CARTESIAN_POINT('Ctrl Pts',(18.6709477710271,16.6503961924556,-20.0363993923192));
#45231=CARTESIAN_POINT('Ctrl Pts',(18.5870183641888,16.6552229364175,-20.0405689590696));
#45232=CARTESIAN_POINT('Ctrl Pts',(18.500138140141,16.6602193806036,-20.0448851207954));
#45233=CARTESIAN_POINT('Ctrl Pts',(18.4135439525353,16.6696490660532,-20.0492012825211));
#45234=CARTESIAN_POINT('Ctrl Pts',(18.3277166966719,16.6834450792442,-20.0535174442468));
#45235=CARTESIAN_POINT('Ctrl Pts',(18.2446852202539,16.696791694284,-20.0576930091876));
#45236=CARTESIAN_POINT('Ctrl Pts',(18.1623719289201,16.7142243989078,-20.0618685741284));
#45237=CARTESIAN_POINT('Ctrl Pts',(18.0812003839193,16.7356308030427,-20.0660441390692));
#45238=CARTESIAN_POINT('Ctrl Pts',(17.9959291092702,16.7581183800159,-20.0704305991874));
#45239=CARTESIAN_POINT('Ctrl Pts',(17.9119185059183,16.7849914459601,-20.0748170593056));
#45240=CARTESIAN_POINT('Ctrl Pts',(17.8296377675515,16.8160618061167,-20.0792035194238));
#45241=CARTESIAN_POINT('Ctrl Pts',(17.7473570291847,16.8471321662734,-20.0835899795421));
#45242=CARTESIAN_POINT('Ctrl Pts',(17.6668066567997,16.8823995182561,-20.0879764396603));
#45243=CARTESIAN_POINT('Ctrl Pts',(17.5884257348687,16.9216202580024,-20.0923628997785));
#45244=CARTESIAN_POINT('Ctrl Pts',(17.5136510990685,16.9590364615644,-20.0965475399908));
#45245=CARTESIAN_POINT('Ctrl Pts',(17.44057234666,17.0001895266255,-20.1007321802031));
#45246=CARTESIAN_POINT('Ctrl Pts',(17.369587760884,17.0449023009683,-20.1049168204155));
#45247=CARTESIAN_POINT('Ctrl Pts',(17.2987042121717,17.0895514326572,-20.1090955043522));
#45248=CARTESIAN_POINT('Ctrl Pts',(17.2299092952701,17.1377499663397,-20.1132741882888));
#45249=CARTESIAN_POINT('Ctrl Pts',(17.1635782312953,17.1892741361949,-20.1174528722255));
#45250=CARTESIAN_POINT('Ctrl Pts',(17.0960583483994,17.241721748316,-20.1217064486519));
#45251=CARTESIAN_POINT('Ctrl Pts',(17.0310919386145,17.2976151655664,-20.1259600250784));
#45252=CARTESIAN_POINT('Ctrl Pts',(16.969045396673,17.3566712135668,-20.1302136015048));
#45253=CARTESIAN_POINT('Ctrl Pts',(16.9082016412034,17.4145824465075,-20.1343847213749));
#45254=CARTESIAN_POINT('Ctrl Pts',(16.8501659076493,17.4755344558904,-20.138555841245));
#45255=CARTESIAN_POINT('Ctrl Pts',(16.7952502349704,17.5392197068402,-20.142726961115));
#45256=CARTESIAN_POINT('Ctrl Pts',(16.7403529897255,17.6028835876472,-20.1468966813293));
#45257=CARTESIAN_POINT('Ctrl Pts',(16.6885740262376,17.6692785404175,-20.1510664015437));
#45258=CARTESIAN_POINT('Ctrl Pts',(16.6401868618722,17.7380619352452,-20.155236121758));
#45259=CARTESIAN_POINT('Ctrl Pts',(16.5918014193961,17.8068428823705,-20.1594056935901));
#45260=CARTESIAN_POINT('Ctrl Pts',(16.5468078000507,17.8780117258147,-20.1635752654222));
#45261=CARTESIAN_POINT('Ctrl Pts',(16.5054369234628,17.9511958033507,-20.1677448372542));
#45262=CARTESIAN_POINT('Ctrl Pts',(16.462611627541,18.0269527134222,-20.1720609930214));
#45263=CARTESIAN_POINT('Ctrl Pts',(16.4236688015505,18.104868733296,-20.1763771487885));
#45264=CARTESIAN_POINT('Ctrl Pts',(16.3888124800775,18.1845032896303,-20.1806933045556));
#45265=CARTESIAN_POINT('Ctrl Pts',(16.3550914981959,18.2615439903646,-20.1848688745605));
#45266=CARTESIAN_POINT('Ctrl Pts',(16.3251950198591,18.3401925369042,-20.1890444445653));
#45267=CARTESIAN_POINT('Ctrl Pts',(16.2992578088608,18.4200319458494,-20.1932200145702));
#45268=CARTESIAN_POINT('Ctrl Pts',(16.2720106919424,18.5039034812422,-20.1976064632185));
#45269=CARTESIAN_POINT('Ctrl Pts',(16.2491334314256,18.5890887659587,-20.2019929118667));
#45270=CARTESIAN_POINT('Ctrl Pts',(16.2307217504257,18.6750914208485,-20.206379360515));
#45271=CARTESIAN_POINT('Ctrl Pts',(16.2123100694257,18.7610940757384,-20.2107658091633));
#45272=CARTESIAN_POINT('Ctrl Pts',(16.198363984864,18.8479135158795,-20.2151522578116));
#45273=CARTESIAN_POINT('Ctrl Pts',(16.1889163328193,18.9350486871749,-20.2195387064599));
#45274=CARTESIAN_POINT('Ctrl Pts',(16.1790436177041,19.0261041916152,-20.2241225075637));
#45275=CARTESIAN_POINT('Ctrl Pts',(16.1740562221026,19.1176988529932,-20.2287063086676));
#45276=CARTESIAN_POINT('Ctrl Pts',(16.17400047263,19.2094444083109,-20.2332901097715));
#45277=CARTESIAN_POINT('Ctrl Pts',(16.1740004726297,19.2094444088938,-20.2332901098006));
#45278=CARTESIAN_POINT('Ctrl Pts',(16.1739502760983,19.2920516545602,-20.2374173417146));
#45279=CARTESIAN_POINT('Ctrl Pts',(16.1779027082651,19.3748187791154,-20.2415445736285));
#45280=CARTESIAN_POINT('Ctrl Pts',(16.1858778001794,19.4573194161684,-20.2456718055424));
#45281=CARTESIAN_POINT('Ctrl Pts',(16.1940130436991,19.5414767876655,-20.249881918359));
#45282=CARTESIAN_POINT('Ctrl Pts',(16.2063343518328,19.6253563595504,-20.2540920311757));
#45283=CARTESIAN_POINT('Ctrl Pts',(16.222807033423,19.7085036528651,-20.2583021439923));
#45284=CARTESIAN_POINT('Ctrl Pts',(16.2389199317254,19.7898349087365,-20.2624203028533));
#45285=CARTESIAN_POINT('Ctrl Pts',(16.2590046102348,19.8704650577792,-20.2665384617144));
#45286=CARTESIAN_POINT('Ctrl Pts',(16.2829763020121,19.9499741753957,-20.2706566205754));
#45287=CARTESIAN_POINT('Ctrl Pts',(16.3069370246241,20.0294469105714,-20.2747728950152));
#45288=CARTESIAN_POINT('Ctrl Pts',(16.334781094809,20.1077991798405,-20.278889169455));
#45289=CARTESIAN_POINT('Ctrl Pts',(16.3663732871992,20.1846240284793,-20.2830054438948));
#45290=CARTESIAN_POINT('Ctrl Pts',(16.3979610861523,20.2614381933028,-20.2871211458959));
#45291=CARTESIAN_POINT('Ctrl Pts',(16.4332957916267,20.3367249220046,-20.291236847897));
#45292=CARTESIAN_POINT('Ctrl Pts',(16.4721937795329,20.4100965853743,-20.2953525498981));
#45293=CARTESIAN_POINT('Ctrl Pts',(16.5126461135564,20.4864001474415,-20.2996327135017));
#45294=CARTESIAN_POINT('Ctrl Pts',(16.5569522565608,20.5606318773211,-20.3039128771053));
#45295=CARTESIAN_POINT('Ctrl Pts',(16.6048536565745,20.6323851864564,-20.3081930407089));
#45296=CARTESIAN_POINT('Ctrl Pts',(16.6509736168395,20.7014700099742,-20.3123140262181));
#45297=CARTESIAN_POINT('Ctrl Pts',(16.700425807859,20.7682571429841,-20.3164350117273));
#45298=CARTESIAN_POINT('Ctrl Pts',(16.7529371454851,20.832416037438,-20.3205559972365));
#45299=CARTESIAN_POINT('Ctrl Pts',(16.8054841275711,20.8966184826611,-20.3246797800521));
#45300=CARTESIAN_POINT('Ctrl Pts',(16.8610940675905,20.9581887928557,-20.3288035628677));
#45301=CARTESIAN_POINT('Ctrl Pts',(16.9194565998598,21.0168328408266,-20.3329273456833));
#45302=CARTESIAN_POINT('Ctrl Pts',(16.9779086865543,21.0755668751946,-20.3370574562401));
#45303=CARTESIAN_POINT('Ctrl Pts',(17.0391214360201,21.1313653808553,-20.3411875667969));
#45304=CARTESIAN_POINT('Ctrl Pts',(17.102751683912,21.1839746402982,-20.3453176773537));
#45305=CARTESIAN_POINT('Ctrl Pts',(17.1099251002331,21.189905595038,-20.3457832892829));
#45306=CARTESIAN_POINT('Ctrl Pts',(17.1171292123955,21.1957960624817,-20.3462489012121));
#45307=CARTESIAN_POINT('Ctrl Pts',(17.1243635072226,21.201645714616,-20.3467145131413));
#45308=CARTESIAN_POINT('Ctrl Pts',(17.189381078246,21.254218934563,-20.3508991582794));
#45309=CARTESIAN_POINT('Ctrl Pts',(17.2570980356913,21.3037012786361,-20.3550838034176));
#45310=CARTESIAN_POINT('Ctrl Pts',(17.3271882231611,21.349803549779,-20.3592684485557));
#45311=CARTESIAN_POINT('Ctrl Pts',(17.3971786443956,21.3958401990397,-20.3634471372781));
#45312=CARTESIAN_POINT('Ctrl Pts',(17.469535204727,21.4385060812658,-20.3676258260006));
#45313=CARTESIAN_POINT('Ctrl Pts',(17.5438988654553,21.477552291379,-20.371804514723));
#45314=CARTESIAN_POINT('Ctrl Pts',(17.619595201075,21.5172982505808,-20.3760580899355));
#45315=CARTESIAN_POINT('Ctrl Pts',(17.6973709112596,21.5532932167484,-20.380311665148));
#45316=CARTESIAN_POINT('Ctrl Pts',(17.7768165359119,21.5853209168257,-20.3845652403605));
#45317=CARTESIAN_POINT('Ctrl Pts',(17.8547221935262,21.6167277947667,-20.3887363646432));
#45318=CARTESIAN_POINT('Ctrl Pts',(17.9342331579704,21.6443196566907,-20.3929074889259));
#45319=CARTESIAN_POINT('Ctrl Pts',(18.0149402978303,21.6679397926517,-20.3970786132086));
#45320=CARTESIAN_POINT('Ctrl Pts',(18.0956203528785,21.6915520018428,-20.401248337688));
#45321=CARTESIAN_POINT('Ctrl Pts',(18.1774953449549,21.711195003098,-20.4054180621675));
#45322=CARTESIAN_POINT('Ctrl Pts',(18.2601401458989,21.7267616816128,-20.409587786647));
#45323=CARTESIAN_POINT('Ctrl Pts',(18.3427820028615,21.7423278056098,-20.4137573625921));
#45324=CARTESIAN_POINT('Ctrl Pts',(18.4261931619307,21.7538178112606,-20.4179269385372));
#45325=CARTESIAN_POINT('Ctrl Pts',(18.5099387942267,21.7611757931694,-20.4220965144823));
#45326=CARTESIAN_POINT('Ctrl Pts',(18.596628364788,21.7687924326811,-20.4264126649273));
#45327=CARTESIAN_POINT('Ctrl Pts',(18.6836758371978,21.7719810786796,-20.4307288153724));
#45328=CARTESIAN_POINT('Ctrl Pts',(18.7705956997404,21.7707384152996,-20.4350449658174));
#45329=CARTESIAN_POINT('Ctrl Pts',(18.854684587927,21.7695362253863,-20.4392205395189));
#45330=CARTESIAN_POINT('Ctrl Pts',(18.9386535840458,21.7641870268945,-20.4433961132204));
#45331=CARTESIAN_POINT('Ctrl Pts',(19.0220673263579,21.7547407917249,-20.4475716869219));
#45332=CARTESIAN_POINT('Ctrl Pts',(19.1096934355566,21.7448175247481,-20.4519581257387));
#45333=CARTESIAN_POINT('Ctrl Pts',(19.1967061584007,21.7303726255243,-20.4563445645555));
#45334=CARTESIAN_POINT('Ctrl Pts',(19.2826140302888,21.7115244741394,-20.4607310033724));
#45335=CARTESIAN_POINT('Ctrl Pts',(19.3685219021768,21.6926763227546,-20.4651174421892));
#45336=CARTESIAN_POINT('Ctrl Pts',(19.4533243836774,21.6694251459735,-20.469503881006));
#45337=CARTESIAN_POINT('Ctrl Pts',(19.5365517912822,21.6419485026034,-20.4738903198228));
#45338=CARTESIAN_POINT('Ctrl Pts',(19.6159350028657,21.6157409796609,-20.4780741531382));
#45339=CARTESIAN_POINT('Ctrl Pts',(19.6941808258861,21.5855921973816,-20.4822579864537));
#45340=CARTESIAN_POINT('Ctrl Pts',(19.7708697961334,21.5516197952393,-20.4864418197691));
#45341=CARTESIAN_POINT('Ctrl Pts',(19.8474630714802,21.5176897849252,-20.4906204323662));
#45342=CARTESIAN_POINT('Ctrl Pts',(19.9225029325766,21.4799458077275,-20.4947990449632));
#45343=CARTESIAN_POINT('Ctrl Pts',(19.9955857715563,21.4385550141369,-20.4989776575603));
#45344=CARTESIAN_POINT('Ctrl Pts',(20.0685856279724,21.3972112180934,-20.5031515255144));
#45345=CARTESIAN_POINT('Ctrl Pts',(20.1396324803964,21.3522290606009,-20.5073253934684));
#45346=CARTESIAN_POINT('Ctrl Pts',(20.2083448689615,21.3038227845106,-20.5114992614224));
#45347=CARTESIAN_POINT('Ctrl Pts',(20.237161086268,21.2835224311109,-20.5132496748265));
#45348=CARTESIAN_POINT('Ctrl Pts',(20.2655670177483,21.2626204215672,-20.5150000882306));
#45349=CARTESIAN_POINT('Ctrl Pts',(20.2935358855687,21.2411349269503,-20.5167505016347));
#45350=CARTESIAN_POINT('',(16.1742339579337,19.2120076676078,-20.1667099326005));
#45351=CARTESIAN_POINT('Ctrl Pts',(16.1778405256925,19.2120194393453,-20.1667105863375));
#45352=CARTESIAN_POINT('Ctrl Pts',(16.17655676437,19.5768333952661,-20.1847914783409));
#45353=CARTESIAN_POINT('Ctrl Pts',(16.4202751262482,20.7953392457516,-20.245264305905));
#45354=CARTESIAN_POINT('Ctrl Pts',(18.140176361079,22.0902446734967,-20.3396938368464));
#45355=CARTESIAN_POINT('Ctrl Pts',(19.7490825166988,21.6517991916634,-20.4160424757843));
#45356=CARTESIAN_POINT('Ctrl Pts',(20.2940726068359,21.241845339799,-20.4499991791617));
#45357=CARTESIAN_POINT('Ctrl Pts',(20.2935358855687,21.2411349269503,-19.6501081158318));
#45358=CARTESIAN_POINT('Ctrl Pts',(20.3602263184528,21.1899037886027,-19.6542777829748));
#45359=CARTESIAN_POINT('Ctrl Pts',(20.424386701975,21.135385296707,-19.6584474501178));
#45360=CARTESIAN_POINT('Ctrl Pts',(20.485686563464,21.0778674787943,-19.6626171172608));
#45361=CARTESIAN_POINT('Ctrl Pts',(20.5470483458354,21.0202915603581,-19.6667909963133));
#45362=CARTESIAN_POINT('Ctrl Pts',(20.6055434979418,20.959710579369,-19.6709648753658));
#45363=CARTESIAN_POINT('Ctrl Pts',(20.6608777148422,20.8964501689592,-19.6751387544183));
#45364=CARTESIAN_POINT('Ctrl Pts',(20.7162388970532,20.833158930669,-19.6793146674735));
#45365=CARTESIAN_POINT('Ctrl Pts',(20.7684357897789,20.7671860230858,-19.6834905805287));
#45366=CARTESIAN_POINT('Ctrl Pts',(20.8172153439539,20.6988890518836,-19.6876664935839));
#45367=CARTESIAN_POINT('Ctrl Pts',(20.8660828483171,20.6304689403294,-19.6918499358661));
#45368=CARTESIAN_POINT('Ctrl Pts',(20.9115204527854,20.5597167799375,-19.6960333781483));
#45369=CARTESIAN_POINT('Ctrl Pts',(20.9533193396094,20.4870178951862,-19.7002168204305));
#45370=CARTESIAN_POINT('Ctrl Pts',(20.9933959851083,20.417314425699,-19.7042278921611));
#45371=CARTESIAN_POINT('Ctrl Pts',(21.0301277549889,20.3458218456753,-19.7082389638917));
#45372=CARTESIAN_POINT('Ctrl Pts',(21.0633723464503,20.2728966388461,-19.7122500356223));
#45373=CARTESIAN_POINT('Ctrl Pts',(21.0980554588848,20.1968158979922,-19.7164346697447));
#45374=CARTESIAN_POINT('Ctrl Pts',(21.1290718315298,20.1188925846168,-19.7206193038671));
#45375=CARTESIAN_POINT('Ctrl Pts',(21.1562228177911,20.0395147077584,-19.7248039379896));
#45376=CARTESIAN_POINT('Ctrl Pts',(21.1833351579832,19.9602498154855,-19.7289826158031));
#45377=CARTESIAN_POINT('Ctrl Pts',(21.2065928926838,19.8795349037292,-19.7331612936167));
#45378=CARTESIAN_POINT('Ctrl Pts',(21.2258445987322,19.7977797676888,-19.7373399714302));
#45379=CARTESIAN_POINT('Ctrl Pts',(21.2454413793552,19.7145592228832,-19.7415935493833));
#45380=CARTESIAN_POINT('Ctrl Pts',(21.2608869019344,19.6302612334801,-19.7458471273363));
#45381=CARTESIAN_POINT('Ctrl Pts',(21.2720739254944,19.5453362808993,-19.7501007052894));
#45382=CARTESIAN_POINT('Ctrl Pts',(21.283044065894,19.4620577709144,-19.7542718189995));
#45383=CARTESIAN_POINT('Ctrl Pts',(21.2899192902207,19.3781768678187,-19.7584429327095));
#45384=CARTESIAN_POINT('Ctrl Pts',(21.2926499549084,19.2941288653065,-19.7626140464196));
#45385=CARTESIAN_POINT('Ctrl Pts',(21.2953797032962,19.2101090658848,-19.7667837604736));
#45386=CARTESIAN_POINT('Ctrl Pts',(21.2939676391619,19.1259227378137,-19.7709534745275));
#45387=CARTESIAN_POINT('Ctrl Pts',(21.2884161370472,19.0420082877982,-19.7751231885815));
#45388=CARTESIAN_POINT('Ctrl Pts',(21.2828648324763,18.958096823782,-19.779292754261));
#45389=CARTESIAN_POINT('Ctrl Pts',(21.2731744140079,18.8744576775594,-19.7834623199405));
#45390=CARTESIAN_POINT('Ctrl Pts',(21.2593992661634,18.7915258691394,-19.78763188562));
#45391=CARTESIAN_POINT('Ctrl Pts',(21.2451397991587,18.7056782688699,-19.791948048677));
#45392=CARTESIAN_POINT('Ctrl Pts',(21.2265031054902,18.620589192361,-19.796264211734));
#45393=CARTESIAN_POINT('Ctrl Pts',(21.2036071461028,18.5367296210585,-19.800580374791));
#45394=CARTESIAN_POINT('Ctrl Pts',(21.1814570231814,18.4556017774482,-19.8047559387253));
#45395=CARTESIAN_POINT('Ctrl Pts',(21.1553210566047,18.3756249996565,-19.8089315026597));
#45396=CARTESIAN_POINT('Ctrl Pts',(21.1253562910671,18.2972083994838,-19.8131070665941));
#45397=CARTESIAN_POINT('Ctrl Pts',(21.09387807017,18.2148311468024,-19.8174935292124));
#45398=CARTESIAN_POINT('Ctrl Pts',(21.0581743347953,18.1341763575253,-19.8218799918307));
#45399=CARTESIAN_POINT('Ctrl Pts',(21.0184823804552,18.0556904079902,-19.8262664544489));
#45400=CARTESIAN_POINT('Ctrl Pts',(20.978790426115,17.9772044584551,-19.8306529170672));
#45401=CARTESIAN_POINT('Ctrl Pts',(20.9351106070445,17.9008878144474,-19.8350393796855));
#45402=CARTESIAN_POINT('Ctrl Pts',(20.8877320902706,17.827150989689,-19.8394258423038));
#45403=CARTESIAN_POINT('Ctrl Pts',(20.8425335350801,17.7568069145607,-19.8436104767382));
#45404=CARTESIAN_POINT('Ctrl Pts',(20.7938009308883,17.6885486380927,-19.8477951111726));
#45405=CARTESIAN_POINT('Ctrl Pts',(20.7417530082953,17.6227532126017,-19.851979745607));
#45406=CARTESIAN_POINT('Ctrl Pts',(20.6897791695079,17.5570514387929,-19.8561584237298));
#45407=CARTESIAN_POINT('Ctrl Pts',(20.6344996686009,17.4938059105141,-19.8603371018527));
#45408=CARTESIAN_POINT('Ctrl Pts',(20.5761771160359,17.4333657650817,-19.8645157799755));
#45409=CARTESIAN_POINT('Ctrl Pts',(20.5168091743242,17.3718422741975,-19.8687693578509));
#45410=CARTESIAN_POINT('Ctrl Pts',(20.4542882752167,17.3132261339225,-19.8730229357263));
#45411=CARTESIAN_POINT('Ctrl Pts',(20.388935154738,17.2578513539384,-19.8772765136017));
#45412=CARTESIAN_POINT('Ctrl Pts',(20.3248490313739,17.2035501215667,-19.8814476276122));
#45413=CARTESIAN_POINT('Ctrl Pts',(20.258039890023,17.1523660019974,-19.8856187416228));
#45414=CARTESIAN_POINT('Ctrl Pts',(20.1888468727061,17.1045763538696,-19.8897898556334));
#45415=CARTESIAN_POINT('Ctrl Pts',(20.1196770738139,17.0568027420471,-19.8939595699839));
#45416=CARTESIAN_POINT('Ctrl Pts',(20.0481253658473,17.0124216007145,-19.8981292843345));
#45417=CARTESIAN_POINT('Ctrl Pts',(19.974561664793,16.9716682345293,-19.9022989986851));
#45418=CARTESIAN_POINT('Ctrl Pts',(19.9010005814933,16.9309163185474,-19.9064685646569));
#45419=CARTESIAN_POINT('Ctrl Pts',(19.8254280502798,16.8937921432249,-19.9106381306288));
#45420=CARTESIAN_POINT('Ctrl Pts',(19.7482392914822,16.8604854479043,-19.9148076966006));
#45421=CARTESIAN_POINT('Ctrl Pts',(19.6683366724246,16.8260077308154,-19.9191238592993));
#45422=CARTESIAN_POINT('Ctrl Pts',(19.5867025423552,16.7956211424271,-19.923440021998));
#45423=CARTESIAN_POINT('Ctrl Pts',(19.5037967719895,16.7694814295536,-19.9277561846968));
#45424=CARTESIAN_POINT('Ctrl Pts',(19.4235916472118,16.7441932147113,-19.93193174891));
#45425=CARTESIAN_POINT('Ctrl Pts',(19.3421969248366,16.7228795141862,-19.9361073131233));
#45426=CARTESIAN_POINT('Ctrl Pts',(19.2600416084997,16.7056297227501,-19.9402828773365));
#45427=CARTESIAN_POINT('Ctrl Pts',(19.1737368242851,16.6875086857435,-19.944669339278));
#45428=CARTESIAN_POINT('Ctrl Pts',(19.0865931685398,16.6738729730806,-19.9490558012194));
#45429=CARTESIAN_POINT('Ctrl Pts',(18.9991144164059,16.6647646718707,-19.9534422631609));
#45430=CARTESIAN_POINT('Ctrl Pts',(18.9116356642721,16.6556563706608,-19.9578287251023));
#45431=CARTESIAN_POINT('Ctrl Pts',(18.8238223991415,16.6510754351692,-19.9622151870438));
#45432=CARTESIAN_POINT('Ctrl Pts',(18.7361763184546,16.6510009250709,-19.9666016489852));
#45433=CARTESIAN_POINT('Ctrl Pts',(18.6525629441496,16.6509298432758,-19.970786284297));
#45434=CARTESIAN_POINT('Ctrl Pts',(18.5687904831981,16.6549593424975,-19.9749709196088));
#45435=CARTESIAN_POINT('Ctrl Pts',(18.4852943718234,16.6631095960553,-19.9791555549207));
#45436=CARTESIAN_POINT('Ctrl Pts',(18.4019171067173,16.6712482487469,-19.9833342339276));
#45437=CARTESIAN_POINT('Ctrl Pts',(18.3188158638134,16.6834959609774,-19.9875129129346));
#45438=CARTESIAN_POINT('Ctrl Pts',(18.2364263585563,16.6998209001864,-19.9916915919416));
#45439=CARTESIAN_POINT('Ctrl Pts',(18.1525601036944,16.7164384476282,-19.9959451695968));
#45440=CARTESIAN_POINT('Ctrl Pts',(18.0694318349784,16.7372808264264,-20.000198747252));
#45441=CARTESIAN_POINT('Ctrl Pts',(17.9874960098034,16.7622591413911,-20.0044523249072));
#45442=CARTESIAN_POINT('Ctrl Pts',(17.9071486482815,16.7867532097475,-20.008623439812));
#45443=CARTESIAN_POINT('Ctrl Pts',(17.8279483681485,16.8152241408411,-20.0127945547168));
#45444=CARTESIAN_POINT('Ctrl Pts',(17.7503119553988,16.847536898763,-20.0169656696216));
#45445=CARTESIAN_POINT('Ctrl Pts',(17.6727015943022,16.8798388138249,-20.0211353848683));
#45446=CARTESIAN_POINT('Ctrl Pts',(17.5966544827469,16.9159798187962,-20.0253051001149));
#45447=CARTESIAN_POINT('Ctrl Pts',(17.5225687033403,16.955776238713,-20.0294748153615));
#45448=CARTESIAN_POINT('Ctrl Pts',(17.4484855602554,16.9955712424854,-20.03364438223));
#45449=CARTESIAN_POINT('Ctrl Pts',(17.3763640154128,17.0390211841318,-20.0378139490985));
#45450=CARTESIAN_POINT('Ctrl Pts',(17.3065775349575,17.0858964481014,-20.041983515967));
#45451=CARTESIAN_POINT('Ctrl Pts',(17.2343374823222,17.1344197654313,-20.0462996776086));
#45452=CARTESIAN_POINT('Ctrl Pts',(17.1646001863695,17.1866134577581,-20.0506158392503));
#45453=CARTESIAN_POINT('Ctrl Pts',(17.0977455244312,17.2421751496943,-20.0549320008919));
#45454=CARTESIAN_POINT('Ctrl Pts',(17.0330686155278,17.295926950746,-20.0591075659941));
#45455=CARTESIAN_POINT('Ctrl Pts',(16.9710897386954,17.3528303455358,-20.0632831310963));
#45456=CARTESIAN_POINT('Ctrl Pts',(16.9121162724547,17.4125729975043,-20.0674586961985));
#45457=CARTESIAN_POINT('Ctrl Pts',(16.8501642398155,17.4753330650506,-20.0718451561099));
#45458=CARTESIAN_POINT('Ctrl Pts',(16.7915295867849,17.5412263087853,-20.0762316160212));
#45459=CARTESIAN_POINT('Ctrl Pts',(16.7365203854446,17.6098519152073,-20.0806180759326));
#45460=CARTESIAN_POINT('Ctrl Pts',(16.6815111841043,17.6784775216292,-20.0850045358439));
#45461=CARTESIAN_POINT('Ctrl Pts',(16.6301277117768,17.7498349754449,-20.0893909957553));
#45462=CARTESIAN_POINT('Ctrl Pts',(16.5826239199814,17.8234910946867,-20.0937774556667));
#45463=CARTESIAN_POINT('Ctrl Pts',(16.5362791661082,17.8953500892742,-20.0980568909977));
#45464=CARTESIAN_POINT('Ctrl Pts',(16.4934601213733,17.96965463442,-20.1023363263287));
#45465=CARTESIAN_POINT('Ctrl Pts',(16.4544271375725,18.0460332344294,-20.1066157616597));
#45466=CARTESIAN_POINT('Ctrl Pts',(16.4154575008457,18.1222878787389,-20.1108882518464));
#45467=CARTESIAN_POINT('Ctrl Pts',(16.3802619050974,18.2006095046636,-20.1151607420331));
#45468=CARTESIAN_POINT('Ctrl Pts',(16.3490570392734,18.2805984339648,-20.1194332322197));
#45469=CARTESIAN_POINT('Ctrl Pts',(16.3179055659637,18.3604504996733,-20.1236984120403));
#45470=CARTESIAN_POINT('Ctrl Pts',(16.2907313869123,18.4419637898502,-20.1279635918609));
#45471=CARTESIAN_POINT('Ctrl Pts',(16.267704287416,18.5247161971242,-20.1322287716815));
#45472=CARTESIAN_POINT('Ctrl Pts',(16.2447004012398,18.6073851827702,-20.1364896518296));
#45473=CARTESIAN_POINT('Ctrl Pts',(16.2258353998839,18.6912903879612,-20.1407505319778));
#45474=CARTESIAN_POINT('Ctrl Pts',(16.2112300227061,18.7759923659696,-20.1450114121259));
#45475=CARTESIAN_POINT('Ctrl Pts',(16.1966372355967,18.8606213295208,-20.1492686193273));
#45476=CARTESIAN_POINT('Ctrl Pts',(16.1862968405217,18.946045274463,-20.1535258265288));
#45477=CARTESIAN_POINT('Ctrl Pts',(16.1802787590545,19.0318134392765,-20.1577830337302));
#45478=CARTESIAN_POINT('Ctrl Pts',(16.1760723590125,19.0917619816882,-20.160758652563));
#45479=CARTESIAN_POINT('Ctrl Pts',(16.1739765481557,19.1518784238251,-20.1637342713957));
#45480=CARTESIAN_POINT('Ctrl Pts',(16.1740001980189,19.2120069046219,-20.1667098902285));
#45481=CARTESIAN_POINT('Origin',(18.734,19.211,1.76670989022852));
#45482=CARTESIAN_POINT('',(20.2935358855687,21.2411349269503,-18.8501886410431));
#45483=CARTESIAN_POINT('',(20.2933494018239,21.240883566784,-18.9165759007818));
#45484=CARTESIAN_POINT('',(20.2935358855687,21.2411349269503,1.76670989022852));
#45485=CARTESIAN_POINT('',(16.1740009418753,19.2131959965388,-19.4332901097715));
#45486=CARTESIAN_POINT('Ctrl Pts',(20.2933494018237,21.2408835667842,-18.9165759007818));
#45487=CARTESIAN_POINT('Ctrl Pts',(20.460481259703,21.1151428689567,-18.9269774804031));
#45488=CARTESIAN_POINT('Ctrl Pts',(21.2286611573496,20.3759974962177,-18.9797709955848));
#45489=CARTESIAN_POINT('Ctrl Pts',(21.6004478661678,18.2379803543616,-19.074956446327));
#45490=CARTESIAN_POINT('Ctrl Pts',(19.4673983208532,16.2740938868786,-19.2021322530084));
#45491=CARTESIAN_POINT('Ctrl Pts',(16.8320816456072,16.9602242617438,-19.3215765971066));
#45492=CARTESIAN_POINT('Ctrl Pts',(16.1790132394519,18.5174132428891,-19.3986290056444));
#45493=CARTESIAN_POINT('Ctrl Pts',(16.1726852608311,19.213184455598,-19.4332894786216));
#45494=CARTESIAN_POINT('Ctrl Pts',(16.1740009418753,19.2131959965388,-19.4332901097715));
#45495=CARTESIAN_POINT('Ctrl Pts',(16.1741094126172,19.3396465587508,-19.4395926510338));
#45496=CARTESIAN_POINT('Ctrl Pts',(16.1835900621655,19.4657089276735,-19.4458951922961));
#45497=CARTESIAN_POINT('Ctrl Pts',(16.2022529884087,19.5902849447293,-19.4521977335585));
#45498=CARTESIAN_POINT('Ctrl Pts',(16.2064836512067,19.6185248420538,-19.4536264444961));
#45499=CARTESIAN_POINT('Ctrl Pts',(16.2111860003675,19.6466884926971,-19.4550551554337));
#45500=CARTESIAN_POINT('Ctrl Pts',(16.2163575306344,19.6747632978648,-19.4564838663713));
#45501=CARTESIAN_POINT('Ctrl Pts',(16.2315047248246,19.7569932189491,-19.4606685004926));
#45502=CARTESIAN_POINT('Ctrl Pts',(16.2507129697403,19.838633291604,-19.4648531346138));
#45503=CARTESIAN_POINT('Ctrl Pts',(16.273922855402,19.9192516802849,-19.4690377687351));
#45504=CARTESIAN_POINT('Ctrl Pts',(16.2970997046635,19.9997553186653,-19.4732164465475));
#45505=CARTESIAN_POINT('Ctrl Pts',(16.3242667547551,20.0792397233557,-19.4773951243598));
#45506=CARTESIAN_POINT('Ctrl Pts',(16.3553134075107,20.1572822489679,-19.4815738021722));
#45507=CARTESIAN_POINT('Ctrl Pts',(16.3869165517625,20.2367236371946,-19.4858273801256));
#45508=CARTESIAN_POINT('Ctrl Pts',(16.4225396637635,20.31467047214,-19.4900809580789));
#45509=CARTESIAN_POINT('Ctrl Pts',(16.4620126245789,20.3906920640265,-19.4943345360323));
#45510=CARTESIAN_POINT('Ctrl Pts',(16.500720321909,20.4652398230115,-19.4985056497412));
#45511=CARTESIAN_POINT('Ctrl Pts',(16.543129704132,20.537935895187,-19.5026767634501));
#45512=CARTESIAN_POINT('Ctrl Pts',(16.5890321382678,20.6083950308112,-19.506847877159));
#45513=CARTESIAN_POINT('Ctrl Pts',(16.6349191694141,20.678830523216,-19.5110175912119));
#45514=CARTESIAN_POINT('Ctrl Pts',(16.6842966737088,20.7470301846918,-19.5151873052647));
#45515=CARTESIAN_POINT('Ctrl Pts',(16.7369115952943,20.8126360085207,-19.5193570193175));
#45516=CARTESIAN_POINT('Ctrl Pts',(16.7895246446383,20.8782394978417,-19.5235265849959));
#45517=CARTESIAN_POINT('Ctrl Pts',(16.845374593747,20.9412489746849,-19.5276961506742));
#45518=CARTESIAN_POINT('Ctrl Pts',(16.9041676934323,21.0013389985813,-19.5318657163526));
#45519=CARTESIAN_POINT('Ctrl Pts',(16.9650278943555,21.0635417221558,-19.5361818794109));
#45520=CARTESIAN_POINT('Ctrl Pts',(17.0290416909492,21.1226154992726,-19.5404980424693));
#45521=CARTESIAN_POINT('Ctrl Pts',(17.0958426218354,21.1782418266103,-19.5448142055276));
#45522=CARTESIAN_POINT('Ctrl Pts',(17.1604675106422,21.2320561248729,-19.5489897694609));
#45523=CARTESIAN_POINT('Ctrl Pts',(17.2277003349656,21.2826438809482,-19.5531653333942));
#45524=CARTESIAN_POINT('Ctrl Pts',(17.2971780335787,21.3297596930302,-19.5573408973275));
#45525=CARTESIAN_POINT('Ctrl Pts',(17.3701649002202,21.3792552227006,-19.5617273599483));
#45526=CARTESIAN_POINT('Ctrl Pts',(17.4456288796132,21.4249185512742,-19.5661138225692));
#45527=CARTESIAN_POINT('Ctrl Pts',(17.5231197837688,21.466519696642,-19.5705002851901));
#45528=CARTESIAN_POINT('Ctrl Pts',(17.6006106879243,21.5081208420097,-19.574886747811));
#45529=CARTESIAN_POINT('Ctrl Pts',(17.6801279596808,21.54565962526,-19.5792732104319));
#45530=CARTESIAN_POINT('Ctrl Pts',(17.7611994326903,21.5789651720923,-19.5836596730527));
#45531=CARTESIAN_POINT('Ctrl Pts',(17.8385406770856,21.6107382772506,-19.587844307487));
#45532=CARTESIAN_POINT('Ctrl Pts',(17.9175841221713,21.6387774071546,-19.5920289419213));
#45533=CARTESIAN_POINT('Ctrl Pts',(17.9979345050497,21.6628987717978,-19.5962135763555));
#45534=CARTESIAN_POINT('Ctrl Pts',(18.0781705190567,21.6869858026501,-19.6003922544782));
#45535=CARTESIAN_POINT('Ctrl Pts',(18.1597093389463,21.7071660136985,-19.6045709326009));
#45536=CARTESIAN_POINT('Ctrl Pts',(18.2421357220941,21.723303630559,-19.6087496107235));
#45537=CARTESIAN_POINT('Ctrl Pts',(18.3260395379464,21.7397305024131,-19.613003188599));
#45538=CARTESIAN_POINT('Ctrl Pts',(18.4108626031778,21.751968244467,-19.6172567664744));
#45539=CARTESIAN_POINT('Ctrl Pts',(18.4961506937664,21.7599267756301,-19.6215103443499));
#45540=CARTESIAN_POINT('Ctrl Pts',(18.5797853091396,21.7677310152159,-19.6256814583602));
#45541=CARTESIAN_POINT('Ctrl Pts',(18.6638666007977,21.7714204401678,-19.6298525723706));
#45542=CARTESIAN_POINT('Ctrl Pts',(18.7479577055539,21.7709619494156,-19.634023686381));
#45543=CARTESIAN_POINT('Ctrl Pts',(18.8320205926795,21.7705036125146,-19.6381934007314));
#45544=CARTESIAN_POINT('Ctrl Pts',(18.9160928267202,21.7659001267025,-19.6423631150818));
#45545=CARTESIAN_POINT('Ctrl Pts',(18.9997364062976,21.7571704896507,-19.6465328294322));
#45546=CARTESIAN_POINT('Ctrl Pts',(19.0833770094289,21.7484411632419,-19.6507023954039));
#45547=CARTESIAN_POINT('Ctrl Pts',(19.1665885309657,21.7355860261267,-19.6548719613755));
#45548=CARTESIAN_POINT('Ctrl Pts',(19.2489383260604,21.7186759201209,-19.6590415273471));
#45549=CARTESIAN_POINT('Ctrl Pts',(19.3341834370069,21.7011712759268,-19.6633576900461));
#45550=CARTESIAN_POINT('Ctrl Pts',(19.4185045808362,21.6793213182574,-19.667673852745));
#45551=CARTESIAN_POINT('Ctrl Pts',(19.501435588217,21.653261783253,-19.6719900154439));
#45552=CARTESIAN_POINT('Ctrl Pts',(19.581665127909,21.6280511344978,-19.6761655796569));
#45553=CARTESIAN_POINT('Ctrl Pts',(19.6605932821676,21.5989011580776,-19.68034114387));
#45554=CARTESIAN_POINT('Ctrl Pts',(19.737817188692,21.5659842996688,-19.684516708083));
#45555=CARTESIAN_POINT('Ctrl Pts',(19.8189414894304,21.5314048897282,-19.6889031700249));
#45556=CARTESIAN_POINT('Ctrl Pts',(19.8981843303166,21.4926683234582,-19.6932896319667));
#45557=CARTESIAN_POINT('Ctrl Pts',(19.9751086547793,21.4500286525705,-19.6976760939086));
#45558=CARTESIAN_POINT('Ctrl Pts',(20.052032979242,21.4073889816829,-19.7020625558505));
#45559=CARTESIAN_POINT('Ctrl Pts',(20.1266383352643,21.3608465778203,-19.7064490177923));
#45560=CARTESIAN_POINT('Ctrl Pts',(20.1985254700751,21.3107059669157,-19.7108354797342));
#45561=CARTESIAN_POINT('Ctrl Pts',(20.2306963153617,21.2882671002084,-19.7127985039785));
#45562=CARTESIAN_POINT('Ctrl Pts',(20.26237935926,21.2650691592041,-19.7147615282228));
#45563=CARTESIAN_POINT('Ctrl Pts',(20.2935358855687,21.2411349269503,-19.7167245524671));
#45564=CARTESIAN_POINT('',(16.1740010149448,19.2087204131752,-19.3667098901939));
#45565=CARTESIAN_POINT('Ctrl Pts',(16.1740010149441,19.2087204138715,-19.3667098902285));
#45566=CARTESIAN_POINT('Ctrl Pts',(16.173926819566,19.2920425969752,-19.3708480242598));
#45567=CARTESIAN_POINT('Ctrl Pts',(16.1779248169782,19.3754486069208,-19.374986158291));
#45568=CARTESIAN_POINT('Ctrl Pts',(16.1859928190663,19.4585063754938,-19.3791242923223));
#45569=CARTESIAN_POINT('Ctrl Pts',(16.1940571655297,19.5415265104593,-19.3832605513584));
#45570=CARTESIAN_POINT('Ctrl Pts',(16.2061878113245,19.6241982519121,-19.3873968103945));
#45571=CARTESIAN_POINT('Ctrl Pts',(16.2223305526748,19.7060925038549,-19.3915330694306));
#45572=CARTESIAN_POINT('Ctrl Pts',(16.2384710163523,19.7879752008633,-19.395668744858));
#45573=CARTESIAN_POINT('Ctrl Pts',(16.2586223602412,19.8690801670325,-19.3998044202854));
#45574=CARTESIAN_POINT('Ctrl Pts',(16.2826791433891,19.9489878440355,-19.4039400957128));
#45575=CARTESIAN_POINT('Ctrl Pts',(16.3067400382207,20.0289091785212,-19.4080764779923));
#45576=CARTESIAN_POINT('Ctrl Pts',(16.3347075604893,20.1076323699276,-19.4122128602718));
#45577=CARTESIAN_POINT('Ctrl Pts',(16.3664266589092,20.1847538059263,-19.4163492425514));
#45578=CARTESIAN_POINT('Ctrl Pts',(16.3981808282506,20.2619605129437,-19.4204901983133));
#45579=CARTESIAN_POINT('Ctrl Pts',(16.4336946710478,20.3375614976538,-19.4246311540753));
#45580=CARTESIAN_POINT('Ctrl Pts',(16.4727655806453,20.4111745292772,-19.4287721098372));
#45581=CARTESIAN_POINT('Ctrl Pts',(16.5118617772824,20.4848352039083,-19.4329157456625));
#45582=CARTESIAN_POINT('Ctrl Pts',(16.5545193804039,20.556504964772,-19.4370593814878));
#45583=CARTESIAN_POINT('Ctrl Pts',(16.6004918491551,20.6258296612236,-19.4412030173131));
#45584=CARTESIAN_POINT('Ctrl Pts',(16.6465392454204,20.6952673454551,-19.4453534065789));
#45585=CARTESIAN_POINT('Ctrl Pts',(16.6959120078414,20.7623519651714,-19.4495037958447));
#45586=CARTESIAN_POINT('Ctrl Pts',(16.7483230702952,20.826762089801,-19.4536541851104));
#45587=CARTESIAN_POINT('Ctrl Pts',(16.7661884610687,20.848717608205,-19.4550689308268));
#45588=CARTESIAN_POINT('Ctrl Pts',(16.7844065661404,20.8703626874017,-19.4564836765431));
#45589=CARTESIAN_POINT('Ctrl Pts',(16.8029650799464,20.891685615317,-19.4578984222595));
#45590=CARTESIAN_POINT('Ctrl Pts',(16.8578587574058,20.9547560712656,-19.4620830566462));
#45591=CARTESIAN_POINT('Ctrl Pts',(16.915947800584,21.0152517076035,-19.466267691033));
#45592=CARTESIAN_POINT('Ctrl Pts',(16.9769612646036,21.0728310563305,-19.4704523254198));
#45593=CARTESIAN_POINT('Ctrl Pts',(17.0378878835037,21.1303284479763,-19.4746310034971));
#45594=CARTESIAN_POINT('Ctrl Pts',(17.1017303233983,21.1849174841133,-19.4788096815744));
#45595=CARTESIAN_POINT('Ctrl Pts',(17.1681782563646,21.2362906623887,-19.4829883596517));
#45596=CARTESIAN_POINT('Ctrl Pts',(17.2358172209073,21.2885846680663,-19.4872419375387));
#45597=CARTESIAN_POINT('Ctrl Pts',(17.306155687672,21.3375460297098,-19.4914955154258));
#45598=CARTESIAN_POINT('Ctrl Pts',(17.3788280009098,21.382890617154,-19.4957490933129));
#45599=CARTESIAN_POINT('Ctrl Pts',(17.4500914193923,21.4273561111915,-19.4999202072833));
#45600=CARTESIAN_POINT('Ctrl Pts',(17.5235985912763,21.46834356131,-19.5040913212538));
#45601=CARTESIAN_POINT('Ctrl Pts',(17.5989738385243,21.5056275542592,-19.5082624352243));
#45602=CARTESIAN_POINT('Ctrl Pts',(17.6743237928747,21.5428990362019,-19.5124321495369));
#45603=CARTESIAN_POINT('Ctrl Pts',(17.7515401656511,21.5764693252641,-19.5166018638495));
#45604=CARTESIAN_POINT('Ctrl Pts',(17.8302229081156,21.6061590694952,-19.5207715781621));
#45605=CARTESIAN_POINT('Ctrl Pts',(17.9089028507052,21.6358477572358,-19.5249411440981));
#45606=CARTESIAN_POINT('Ctrl Pts',(17.9890486285244,21.6616560130853,-19.5291107100341));
#45607=CARTESIAN_POINT('Ctrl Pts',(18.0702417419437,21.6834532300656,-19.5332802759701));
#45608=CARTESIAN_POINT('Ctrl Pts',(18.1542895053988,21.7060168103939,-19.5375964387177));
#45609=CARTESIAN_POINT('Ctrl Pts',(18.2394591140179,21.724281910891,-19.5419126014652));
#45610=CARTESIAN_POINT('Ctrl Pts',(18.3252730114509,21.7381609067947,-19.5462287642128));
#45611=CARTESIAN_POINT('Ctrl Pts',(18.4082915298627,21.751587795812,-19.5504043283958));
#45612=CARTESIAN_POINT('Ctrl Pts',(18.4919125329025,21.7609099414411,-19.5545798925789));
#45613=CARTESIAN_POINT('Ctrl Pts',(18.5756985998726,21.7661009112592,-19.5587554567619));
#45614=CARTESIAN_POINT('Ctrl Pts',(18.6637165024322,21.7715540646553,-19.5631419187917));
#45615=CARTESIAN_POINT('Ctrl Pts',(18.7519159980506,21.7724477372193,-19.5675283808216));
#45616=CARTESIAN_POINT('Ctrl Pts',(18.8397925195448,21.7688131172563,-19.5719148428514));
#45617=CARTESIAN_POINT('Ctrl Pts',(18.9276690410391,21.7651784972933,-19.5763013048812));
#45618=CARTESIAN_POINT('Ctrl Pts',(19.0152220177587,21.7570157144011,-19.5806877669111));
#45619=CARTESIAN_POINT('Ctrl Pts',(19.1019580505816,21.7444180217667,-19.5850742289409));
#45620=CARTESIAN_POINT('Ctrl Pts',(19.1847019893298,21.732400147836,-19.5892588006086));
#45621=CARTESIAN_POINT('Ctrl Pts',(19.2670105160923,21.7163018984399,-19.5934433722763));
#45622=CARTESIAN_POINT('Ctrl Pts',(19.3484498725015,21.6961662628852,-19.5976279439439));
#45623=CARTESIAN_POINT('Ctrl Pts',(19.4335631521515,21.6751222608761,-19.6020012916013));
#45624=CARTESIAN_POINT('Ctrl Pts',(19.5177264866766,21.6496679803991,-19.6063746392586));
#45625=CARTESIAN_POINT('Ctrl Pts',(19.600451164542,21.6199131116468,-19.6107479869159));
#45626=CARTESIAN_POINT('Ctrl Pts',(19.6793978228884,21.5915171418087,-19.614921604659));
#45627=CARTESIAN_POINT('Ctrl Pts',(19.7570338492619,21.5592049408122,-19.6190952224021));
#45628=CARTESIAN_POINT('Ctrl Pts',(19.8329471632924,21.5231235114698,-19.6232688401453));
#45629=CARTESIAN_POINT('Ctrl Pts',(19.908808933188,21.4870665809402,-19.6274396240572));
#45630=CARTESIAN_POINT('Ctrl Pts',(19.9829499000485,21.4472457028666,-19.6316104079691));
#45631=CARTESIAN_POINT('Ctrl Pts',(20.0549778814522,21.403855999995,-19.6357811918811));
#45632=CARTESIAN_POINT('Ctrl Pts',(20.1269801303178,21.3604817984211,-19.6399504857491));
#45633=CARTESIAN_POINT('Ctrl Pts',(20.1968705003484,21.3135415429754,-19.6441197796171));
#45634=CARTESIAN_POINT('Ctrl Pts',(20.2642825292425,21.2632756590417,-19.6482890734851));
#45635=CARTESIAN_POINT('Ctrl Pts',(20.2740863744592,21.2559654066454,-19.648895420934));
#45636=CARTESIAN_POINT('Ctrl Pts',(20.283837851539,21.2485848909344,-19.6495017683829));
#45637=CARTESIAN_POINT('Ctrl Pts',(20.2935358855687,21.2411349269503,-19.6501081158318));
#45638=CARTESIAN_POINT('Ctrl Pts',(20.2935358855687,21.2411349269503,-18.8501886410431));
#45639=CARTESIAN_POINT('Ctrl Pts',(20.3600880965346,21.190009969743,-18.8543616962283));
#45640=CARTESIAN_POINT('Ctrl Pts',(20.4241919562629,21.1355565384397,-18.8585347514134));
#45641=CARTESIAN_POINT('Ctrl Pts',(20.4855007784819,21.0780417839398,-18.8627078065986));
#45642=CARTESIAN_POINT('Ctrl Pts',(20.5467748064481,21.0205596704667,-18.8668784934731));
#45643=CARTESIAN_POINT('Ctrl Pts',(20.6052566115097,20.9600199972293,-18.8710491803476));
#45644=CARTESIAN_POINT('Ctrl Pts',(20.6606332957843,20.8967295582552,-18.8752198672221));
#45645=CARTESIAN_POINT('Ctrl Pts',(20.7159951643049,20.8334560523205,-18.8793894382502));
#45646=CARTESIAN_POINT('Ctrl Pts',(20.7682532594284,20.7674335885141,-18.8835590092783));
#45647=CARTESIAN_POINT('Ctrl Pts',(20.8171331635652,20.6990041071365,-18.8877285803065));
#45648=CARTESIAN_POINT('Ctrl Pts',(20.8660146528381,20.6305724066455,-18.8918982865505));
#45649=CARTESIAN_POINT('Ctrl Pts',(20.911517467248,20.5597339086927,-18.8960679927945));
#45650=CARTESIAN_POINT('Ctrl Pts',(20.9534097480727,20.4868606390041,-18.9002376990385));
#45651=CARTESIAN_POINT('Ctrl Pts',(20.9953447652096,20.4139130278199,-18.9044116589985));
#45652=CARTESIAN_POINT('Ctrl Pts',(21.0336616621183,20.338926898568,-18.9085856189586));
#45653=CARTESIAN_POINT('Ctrl Pts',(21.0681741689714,20.2622996475347,-18.9127595789187));
#45654=CARTESIAN_POINT('Ctrl Pts',(21.1027039955892,20.1856339418634,-18.9169356335398));
#45655=CARTESIAN_POINT('Ctrl Pts',(21.133425461192,20.1073259026731,-18.9211116881609));
#45656=CARTESIAN_POINT('Ctrl Pts',(21.1602010975522,20.0277914263976,-18.9252877427821));
#45657=CARTESIAN_POINT('Ctrl Pts',(21.1870245425827,19.9481149390228,-18.929471253869));
#45658=CARTESIAN_POINT('Ctrl Pts',(21.2098879562465,19.8672080828444,-18.9336547649561));
#45659=CARTESIAN_POINT('Ctrl Pts',(21.2287042779432,19.7855002746841,-18.9378382760431));
#45660=CARTESIAN_POINT('Ctrl Pts',(21.2457310804045,19.7115632570501,-18.9416239158733));
#45661=CARTESIAN_POINT('Ctrl Pts',(21.2594446080859,19.6369707745906,-18.9454095557035));
#45662=CARTESIAN_POINT('Ctrl Pts',(21.2698170137415,19.5620442604844,-18.9491951955337));
#45663=CARTESIAN_POINT('Ctrl Pts',(21.2812826384042,19.4792207269144,-18.9533798299225));
#45664=CARTESIAN_POINT('Ctrl Pts',(21.2887076244829,19.3956807451278,-18.9575644643113));
#45665=CARTESIAN_POINT('Ctrl Pts',(21.2920126435715,19.3118529391169,-18.9617490987001));
#45666=CARTESIAN_POINT('Ctrl Pts',(21.2953129583745,19.228144451612,-18.9659277767799));
#45667=CARTESIAN_POINT('Ctrl Pts',(21.294504936491,19.1441494093845,-18.9701064548596));
#45668=CARTESIAN_POINT('Ctrl Pts',(21.2895607321101,19.0603038006549,-18.9742851329393));
#45669=CARTESIAN_POINT('Ctrl Pts',(21.2845279064127,18.9749553195403,-18.9785387108258));
#45670=CARTESIAN_POINT('Ctrl Pts',(21.2752090914542,18.8897621593927,-18.9827922887123));
#45671=CARTESIAN_POINT('Ctrl Pts',(21.2616304174303,18.8051866526579,-18.9870458665988));
#45672=CARTESIAN_POINT('Ctrl Pts',(21.2483149925156,18.7222508072601,-18.9912169805726));
#45673=CARTESIAN_POINT('Ctrl Pts',(21.2309034822292,18.6399093552897,-18.9953880945464));
#45674=CARTESIAN_POINT('Ctrl Pts',(21.2094728610011,18.5585935971749,-18.9995592085202));
#45675=CARTESIAN_POINT('Ctrl Pts',(21.1880494310247,18.4773051253474,-19.0037289228364));
#45676=CARTESIAN_POINT('Ctrl Pts',(21.1626096856898,18.3970421082987,-19.0078986371526));
#45677=CARTESIAN_POINT('Ctrl Pts',(21.1332813336496,18.3182239463334,-19.0120683514689));
#45678=CARTESIAN_POINT('Ctrl Pts',(21.1039540252378,18.2394085890558,-19.0162379174088));
#45679=CARTESIAN_POINT('Ctrl Pts',(21.0707385464732,18.1620384154915,-19.0204074833488));
#45680=CARTESIAN_POINT('Ctrl Pts',(21.0338114728017,18.0865147001541,-19.0245770492887));
#45681=CARTESIAN_POINT('Ctrl Pts',(20.9955860886931,18.0083356639876,-19.0288932120326));
#45682=CARTESIAN_POINT('Ctrl Pts',(20.9533834858384,17.9321358186686,-19.0332093747765));
#45683=CARTESIAN_POINT('Ctrl Pts',(20.9074514472649,17.8583327066931,-19.0375255375203));
#45684=CARTESIAN_POINT('Ctrl Pts',(20.8630156401098,17.7869337234772,-19.041701101708));
#45685=CARTESIAN_POINT('Ctrl Pts',(20.8150899458169,17.7177780846045,-19.0458766658958));
#45686=CARTESIAN_POINT('Ctrl Pts',(20.7639418957711,17.6512128671536,-19.0500522300835));
#45687=CARTESIAN_POINT('Ctrl Pts',(20.7102104791443,17.5812855985968,-19.0544386921054));
#45688=CARTESIAN_POINT('Ctrl Pts',(20.6529230087042,17.5142177570107,-19.0588251541274));
#45689=CARTESIAN_POINT('Ctrl Pts',(20.5924345734847,17.4503691653055,-19.0632116161493));
#45690=CARTESIAN_POINT('Ctrl Pts',(20.5319461382652,17.3865205736004,-19.0675980781713));
#45691=CARTESIAN_POINT('Ctrl Pts',(20.468257210959,17.3258915767387,-19.0719845401932));
#45692=CARTESIAN_POINT('Ctrl Pts',(20.4017623229458,17.2687927931958,-19.0763710022152));
#45693=CARTESIAN_POINT('Ctrl Pts',(20.3383269634738,17.2143212094742,-19.0805556366057));
#45694=CARTESIAN_POINT('Ctrl Pts',(20.2721020634018,17.1628593635266,-19.0847402709962));
#45695=CARTESIAN_POINT('Ctrl Pts',(20.2034050887144,17.114705964026,-19.0889249053867));
#45696=CARTESIAN_POINT('Ctrl Pts',(20.1348058956684,17.0666211049301,-19.093103583468));
#45697=CARTESIAN_POINT('Ctrl Pts',(20.0637419907199,17.0218356001937,-19.0972822615494));
#45698=CARTESIAN_POINT('Ctrl Pts',(19.9905648985565,16.9806088558919,-19.1014609396307));
#45699=CARTESIAN_POINT('Ctrl Pts',(19.91607615955,16.9386431517953,-19.1057145175168));
#45700=CARTESIAN_POINT('Ctrl Pts',(19.8393980962005,16.900365358686,-19.1099680954029));
#45701=CARTESIAN_POINT('Ctrl Pts',(19.7609336007079,16.8660037569887,-19.114221673289));
#45702=CARTESIAN_POINT('Ctrl Pts',(19.6839902926328,16.8323083220184,-19.1183927872642));
#45703=CARTESIAN_POINT('Ctrl Pts',(19.6053296420405,16.8023787805159,-19.1225639012394));
#45704=CARTESIAN_POINT('Ctrl Pts',(19.5253559691354,16.7763838639092,-19.1267350152147));
#45705=CARTESIAN_POINT('Ctrl Pts',(19.4454091321692,16.7503976701479,-19.1309047295323));
#45706=CARTESIAN_POINT('Ctrl Pts',(19.3641505850606,16.7283436212314,-19.13507444385));
#45707=CARTESIAN_POINT('Ctrl Pts',(19.2820021033662,16.7103413478233,-19.1392441581676));
#45708=CARTESIAN_POINT('Ctrl Pts',(19.1998565448679,16.6923397150134,-19.1434137241089));
#45709=CARTESIAN_POINT('Ctrl Pts',(19.1168215642988,16.6783896686896,-19.1475832900501));
#45710=CARTESIAN_POINT('Ctrl Pts',(19.0333301469618,16.6685599391294,-19.1517528559914));
#45711=CARTESIAN_POINT('Ctrl Pts',(18.9469032742682,16.6583846083898,-19.1560690187335));
#45712=CARTESIAN_POINT('Ctrl Pts',(18.8599877947896,16.6526247876704,-19.1603851814756));
#45713=CARTESIAN_POINT('Ctrl Pts',(18.77306891594,16.651298138492,-19.1647013442177));
#45714=CARTESIAN_POINT('Ctrl Pts',(18.6889814105451,16.650014704773,-19.1688769084066));
#45715=CARTESIAN_POINT('Ctrl Pts',(18.6048911930079,16.652879993597,-19.1730524725954));
#45716=CARTESIAN_POINT('Ctrl Pts',(18.5212349098901,16.6598569196475,-19.1772280367843));
#45717=CARTESIAN_POINT('Ctrl Pts',(18.4333533466031,16.667186233662,-19.181614498803));
#45718=CARTESIAN_POINT('Ctrl Pts',(18.345951284399,16.6790533797553,-19.1860009608217));
#45719=CARTESIAN_POINT('Ctrl Pts',(18.2595234803602,16.6953545495618,-19.1903874228404));
#45720=CARTESIAN_POINT('Ctrl Pts',(18.1730956763213,16.7116557193683,-19.1947738848591));
#45721=CARTESIAN_POINT('Ctrl Pts',(18.0876426763664,16.7323907021497,-19.1991603468778));
#45722=CARTESIAN_POINT('Ctrl Pts',(18.0036392138284,16.7573958913421,-19.2035468088965));
#45723=CARTESIAN_POINT('Ctrl Pts',(17.9235008748349,16.7812505547995,-19.2077314433106));
#45724=CARTESIAN_POINT('Ctrl Pts',(17.8443833236132,16.8090798944622,-19.2119160777247));
#45725=CARTESIAN_POINT('Ctrl Pts',(17.7667095652053,16.8407786570123,-19.2161007121388));
#45726=CARTESIAN_POINT('Ctrl Pts',(17.6891463657766,16.8724323002981,-19.2202793902438));
#45727=CARTESIAN_POINT('Ctrl Pts',(17.6130232994518,16.9079442542207,-19.2244580683488));
#45728=CARTESIAN_POINT('Ctrl Pts',(17.5387487593373,16.9471593537322,-19.2286367464538));
#45729=CARTESIAN_POINT('Ctrl Pts',(17.4631429019463,16.9870773554683,-19.232890324334));
#45730=CARTESIAN_POINT('Ctrl Pts',(17.3894529543325,17.0308324287606,-19.2371439022142));
#45731=CARTESIAN_POINT('Ctrl Pts',(17.3180889421074,17.0782093688931,-19.2413974800944));
#45732=CARTESIAN_POINT('Ctrl Pts',(17.2481084600744,17.1246678148849,-19.2455685940934));
#45733=CARTESIAN_POINT('Ctrl Pts',(17.1803649335802,17.1746086808986,-19.2497397080924));
#45734=CARTESIAN_POINT('Ctrl Pts',(17.1152190899139,17.2277833287458,-19.2539108220915));
#45735=CARTESIAN_POINT('Ctrl Pts',(17.0500951065651,17.2809401333258,-19.2580805364329));
#45736=CARTESIAN_POINT('Ctrl Pts',(16.9875674309667,17.337328274007,-19.2622502507743));
#45737=CARTESIAN_POINT('Ctrl Pts',(16.9279649526866,17.3966578580996,-19.2664199651157));
#45738=CARTESIAN_POINT('Ctrl Pts',(16.8683645953195,17.45598533099,-19.2705895310807));
#45739=CARTESIAN_POINT('Ctrl Pts',(16.8116895537474,17.5182537140333,-19.2747590970458));
#45740=CARTESIAN_POINT('Ctrl Pts',(16.7582319859915,17.5831361375039,-19.2789286630108));
#45741=CARTESIAN_POINT('Ctrl Pts',(16.702894916699,17.6502997462159,-19.2832448257247));
#45742=CARTESIAN_POINT('Ctrl Pts',(16.6510061189344,17.7202642276924,-19.2875609884387));
#45743=CARTESIAN_POINT('Ctrl Pts',(16.6028430768051,17.7926311591414,-19.2918771511526));
#45744=CARTESIAN_POINT('Ctrl Pts',(16.556248940208,17.8626407461605,-19.2960527153649));
#45745=CARTESIAN_POINT('Ctrl Pts',(16.5131417547257,17.9348982385108,-19.3002282795771));
#45746=CARTESIAN_POINT('Ctrl Pts',(16.4737266859811,18.0090164119531,-19.3044038437894));
#45747=CARTESIAN_POINT('Ctrl Pts',(16.4323208564697,18.086878116905,-19.3087903057542));
#45748=CARTESIAN_POINT('Ctrl Pts',(16.3949901703488,18.1667928797147,-19.3131767677189));
#45749=CARTESIAN_POINT('Ctrl Pts',(16.3619151438302,18.2482884984951,-19.3175632296837));
#45750=CARTESIAN_POINT('Ctrl Pts',(16.3288401173116,18.3297841172754,-19.3219496916485));
#45751=CARTESIAN_POINT('Ctrl Pts',(16.3000208686933,18.4128600189268,-19.3263361536133));
#45752=CARTESIAN_POINT('Ctrl Pts',(16.2755767948946,18.4970284707363,-19.330722615578));
#45753=CARTESIAN_POINT('Ctrl Pts',(16.2465257453506,18.5970601546401,-19.3359357942368));
#45754=CARTESIAN_POINT('Ctrl Pts',(16.2235642356451,18.6989346521906,-19.3411489728956));
#45755=CARTESIAN_POINT('Ctrl Pts',(16.2068848499389,18.8019901977558,-19.3463621515544));
#45756=CARTESIAN_POINT('Ctrl Pts',(16.1904712789818,18.9034033756426,-19.3514922492292));
#45757=CARTESIAN_POINT('Ctrl Pts',(16.1801412136981,19.0059603454969,-19.356622346904));
#45758=CARTESIAN_POINT('Ctrl Pts',(16.1760324691886,19.1090092586819,-19.3617524445787));
#45759=CARTESIAN_POINT('Ctrl Pts',(16.1747089805831,19.1422028685768,-19.3634049264505));
#45760=CARTESIAN_POINT('Ctrl Pts',(16.1740306434087,19.1754473495068,-19.3650574083222));
#45761=CARTESIAN_POINT('Ctrl Pts',(16.1740010149447,19.2087204131752,-19.3667098901939));
#45762=CARTESIAN_POINT('Origin',(18.734,19.211,1.76670989022852));
#45763=CARTESIAN_POINT('',(20.2935358855687,21.2411349269503,-18.0500683201495));
#45764=CARTESIAN_POINT('',(20.2935358855687,21.2411349269503,-18.1167065565846));
#45765=CARTESIAN_POINT('',(20.2935358855687,21.2411349269503,1.76670989022852));
#45766=CARTESIAN_POINT('',(16.1743944470979,19.2113823947302,-18.633290134885));
#45767=CARTESIAN_POINT('Ctrl Pts',(20.2935358855687,21.2411349269503,-18.1167065565846));
#45768=CARTESIAN_POINT('Ctrl Pts',(20.3602206228857,21.1899081638987,-18.1208760360078));
#45769=CARTESIAN_POINT('Ctrl Pts',(20.4243870798335,21.1353858945908,-18.125045515431));
#45770=CARTESIAN_POINT('Ctrl Pts',(20.4857019867477,21.0778530069677,-18.1292149948543));
#45771=CARTESIAN_POINT('Ctrl Pts',(20.5470276395309,21.020310036301,-18.1333852050081));
#45772=CARTESIAN_POINT('Ctrl Pts',(20.6055004154035,20.9597557153283,-18.137555415162));
#45773=CARTESIAN_POINT('Ctrl Pts',(20.660823359764,20.896512307955,-18.1417256253158));
#45774=CARTESIAN_POINT('Ctrl Pts',(20.7162074113154,20.83319904481,-18.1459004416928));
#45775=CARTESIAN_POINT('Ctrl Pts',(20.7684343845667,20.7671911142531,-18.1500752580698));
#45776=CARTESIAN_POINT('Ctrl Pts',(20.8172475167671,20.698844005225,-18.1542500744469));
#45777=CARTESIAN_POINT('Ctrl Pts',(20.8660913973001,20.6304538430357,-18.1584275206212));
#45778=CARTESIAN_POINT('Ctrl Pts',(20.9115169082914,20.5597219564181,-18.1626049667955));
#45779=CARTESIAN_POINT('Ctrl Pts',(20.953311843756,20.4870309322914,-18.1667824129698));
#45780=CARTESIAN_POINT('Ctrl Pts',(20.9951752878851,20.4142207558097,-18.1709667066546));
#45781=CARTESIAN_POINT('Ctrl Pts',(21.0333960698403,20.3394454413685,-18.1751510003393));
#45782=CARTESIAN_POINT('Ctrl Pts',(21.0678091422995,20.2631097315961,-18.1793352940241));
#45783=CARTESIAN_POINT('Ctrl Pts',(21.0825869336838,20.2303293631612,-18.1811321292017));
#45784=CARTESIAN_POINT('Ctrl Pts',(21.0966631839603,20.1972614661371,-18.1829289643794));
#45785=CARTESIAN_POINT('Ctrl Pts',(21.1100276507034,20.1639389293617,-18.184725799557));
#45786=CARTESIAN_POINT('Ctrl Pts',(21.1411520453503,20.0863343526005,-18.1889104339505));
#45787=CARTESIAN_POINT('Ctrl Pts',(21.1685283427045,20.00705890033,-18.193095068344));
#45788=CARTESIAN_POINT('Ctrl Pts',(21.1919760688457,19.926509360513,-18.1972797027374));
#45789=CARTESIAN_POINT('Ctrl Pts',(21.2153904200511,19.8460744729958,-18.2014583808218));
#45790=CARTESIAN_POINT('Ctrl Pts',(21.2348871797096,19.7643695380467,-18.2056370589062));
#45791=CARTESIAN_POINT('Ctrl Pts',(21.2503340551361,19.6818109206064,-18.2098157369906));
#45792=CARTESIAN_POINT('Ctrl Pts',(21.266057804701,19.5977724992935,-18.2140693148759));
#45793=CARTESIAN_POINT('Ctrl Pts',(21.2775848741471,19.5128499374384,-18.2183228927613));
#45794=CARTESIAN_POINT('Ctrl Pts',(21.2848289888802,19.4274981974251,-18.2225764706466));
#45795=CARTESIAN_POINT('Ctrl Pts',(21.2919326623144,19.3438011674312,-18.226747584625));
#45796=CARTESIAN_POINT('Ctrl Pts',(21.2949179252555,19.2596919311855,-18.2309186986034));
#45797=CARTESIAN_POINT('Ctrl Pts',(21.2937553357682,19.1756076137218,-18.2350898125818));
#45798=CARTESIAN_POINT('Ctrl Pts',(21.2925931363989,19.0915515115629,-18.2392595269026));
#45799=CARTESIAN_POINT('Ctrl Pts',(21.287285855196,19.0075207711856,-18.2434292412234));
#45800=CARTESIAN_POINT('Ctrl Pts',(21.2778561566697,18.9239532195377,-18.2475989555442));
#45801=CARTESIAN_POINT('Ctrl Pts',(21.2684267936926,18.8403886415822,-18.2517685214887));
#45802=CARTESIAN_POINT('Ctrl Pts',(21.2548753574853,18.7572876766215,-18.2559380874332));
#45803=CARTESIAN_POINT('Ctrl Pts',(21.2372763100334,18.6750823611547,-18.2601076533776));
#45804=CARTESIAN_POINT('Ctrl Pts',(21.2190585017879,18.5899868082263,-18.264423816116));
#45805=CARTESIAN_POINT('Ctrl Pts',(21.1965032689153,18.5058515744425,-18.2687399788544));
#45806=CARTESIAN_POINT('Ctrl Pts',(21.1697502461669,18.4231416762528,-18.2730561415928));
#45807=CARTESIAN_POINT('Ctrl Pts',(21.143868700315,18.3431260442794,-18.2772317057849));
#45808=CARTESIAN_POINT('Ctrl Pts',(21.114058861765,18.2644447370881,-18.281407269977));
#45809=CARTESIAN_POINT('Ctrl Pts',(21.0804965434245,18.1874991589174,-18.2855828341691));
#45810=CARTESIAN_POINT('Ctrl Pts',(21.045239072183,18.1066672425405,-18.2899692961807));
#45811=CARTESIAN_POINT('Ctrl Pts',(21.0058403441653,18.0277515290332,-18.2943557581922));
#45812=CARTESIAN_POINT('Ctrl Pts',(20.9625580617871,17.9511869324206,-18.2987422202038));
#45813=CARTESIAN_POINT('Ctrl Pts',(20.9192757794088,17.8746223358079,-18.3031286822153));
#45814=CARTESIAN_POINT('Ctrl Pts',(20.8721103180847,17.8004093049791,-18.3075151442269));
#45815=CARTESIAN_POINT('Ctrl Pts',(20.8213695361433,17.7289445288449,-18.3119016062384));
#45816=CARTESIAN_POINT('Ctrl Pts',(20.7729634127898,17.6607679529896,-18.3160862406309));
#45817=CARTESIAN_POINT('Ctrl Pts',(20.7211235735797,17.5948385205844,-18.3202708750235));
#45818=CARTESIAN_POINT('Ctrl Pts',(20.6660859672865,17.5315227554341,-18.324455509416));
#45819=CARTESIAN_POINT('Ctrl Pts',(20.6111267002136,17.4682971124387,-18.3286341874995));
#45820=CARTESIAN_POINT('Ctrl Pts',(20.5529790062397,17.407678091374,-18.3328128655829));
#45821=CARTESIAN_POINT('Ctrl Pts',(20.491921374867,17.3500022998978,-18.3369915436664));
#45822=CARTESIAN_POINT('Ctrl Pts',(20.4297693293241,17.2912927113015,-18.3412451215519));
#45823=CARTESIAN_POINT('Ctrl Pts',(20.3646022781507,17.23563329804,-18.3454986994375));
#45824=CARTESIAN_POINT('Ctrl Pts',(20.2967560739111,17.1833428659031,-18.349752277323));
#45825=CARTESIAN_POINT('Ctrl Pts',(20.2302252007414,17.1320661858371,-18.3539233913005));
#45826=CARTESIAN_POINT('Ctrl Pts',(20.1611185098597,17.0840293178159,-18.358094505278));
#45827=CARTESIAN_POINT('Ctrl Pts',(20.0897876178817,17.0394936253378,-18.3622656192554));
#45828=CARTESIAN_POINT('Ctrl Pts',(20.0184806616734,16.9949728772414,-18.3664353335753));
#45829=CARTESIAN_POINT('Ctrl Pts',(19.9449513765316,16.9539512148436,-18.3706050478952));
#45830=CARTESIAN_POINT('Ctrl Pts',(19.8695801735014,16.9166465683006,-18.3747747622151));
#45831=CARTESIAN_POINT('Ctrl Pts',(19.7942116525019,16.8793432492171,-18.3789443281586));
#45832=CARTESIAN_POINT('Ctrl Pts',(19.7170017566051,16.8457568863073,-18.3831138941022));
#45833=CARTESIAN_POINT('Ctrl Pts',(19.6383540649958,16.816058721988,-18.3872834600458));
#45834=CARTESIAN_POINT('Ctrl Pts',(19.5569412175515,16.7853164068402,-18.3915996227853));
#45835=CARTESIAN_POINT('Ctrl Pts',(19.473988080848,16.7587409819329,-18.3959157855248));
#45836=CARTESIAN_POINT('Ctrl Pts',(19.3899612417722,16.7364667411221,-18.4002319482643));
#45837=CARTESIAN_POINT('Ctrl Pts',(19.3086715681611,16.7149180813683,-18.4044075124555));
#45838=CARTESIAN_POINT('Ctrl Pts',(19.2263775401993,16.6973947388031,-18.4085830766467));
#45839=CARTESIAN_POINT('Ctrl Pts',(19.1435118395199,16.6839661550955,-18.4127586408379));
#45840=CARTESIAN_POINT('Ctrl Pts',(19.0564607892622,16.6698593255431,-18.4171451028516));
#45841=CARTESIAN_POINT('Ctrl Pts',(18.9687793786238,16.6602718418454,-18.4215315648652));
#45842=CARTESIAN_POINT('Ctrl Pts',(18.880972790904,16.6552224277661,-18.4259180268789));
#45843=CARTESIAN_POINT('Ctrl Pts',(18.7931662031841,16.6501730136867,-18.4303044888925));
#45844=CARTESIAN_POINT('Ctrl Pts',(18.7052350190325,16.6496615965365,-18.4346909509062));
#45845=CARTESIAN_POINT('Ctrl Pts',(18.6176794289206,16.6536440363642,-18.4390774129198));
#45846=CARTESIAN_POINT('Ctrl Pts',(18.5341524013311,16.6574432382304,-18.4432620473123));
#45847=CARTESIAN_POINT('Ctrl Pts',(18.4506562604971,16.6653459878634,-18.4474466817047));
#45848=CARTESIAN_POINT('Ctrl Pts',(18.3676269095308,16.6773522820684,-18.4516313160972));
#45849=CARTESIAN_POINT('Ctrl Pts',(18.2847157405689,16.6893414867996,-18.4558099941805));
#45850=CARTESIAN_POINT('Ctrl Pts',(18.2022704931355,16.7054225689873,-18.4599886722639));
#45851=CARTESIAN_POINT('Ctrl Pts',(18.1207249420869,16.725543562373,-18.4641673503472));
#45852=CARTESIAN_POINT('Ctrl Pts',(18.0377177456267,16.746025210108,-18.4684209282328));
#45853=CARTESIAN_POINT('Ctrl Pts',(17.9556432985583,16.7706930025008,-18.4726745061184));
#45854=CARTESIAN_POINT('Ctrl Pts',(17.8749514567222,16.7994371042222,-18.476928084004));
#45855=CARTESIAN_POINT('Ctrl Pts',(17.7958239837115,16.8276239454371,-18.4810991979813));
#45856=CARTESIAN_POINT('Ctrl Pts',(17.7180264386455,16.8597302905275,-18.4852703119587));
#45857=CARTESIAN_POINT('Ctrl Pts',(17.6419689102697,16.8956019566687,-18.489441425936));
#45858=CARTESIAN_POINT('Ctrl Pts',(17.5659369037323,16.9314615857258,-18.4936111402558));
#45859=CARTESIAN_POINT('Ctrl Pts',(17.491644170023,16.9710838304477,-18.4977808545755));
#45860=CARTESIAN_POINT('Ctrl Pts',(17.4194798631985,17.0142667868074,-18.5019505688953));
#45861=CARTESIAN_POINT('Ctrl Pts',(17.3473181242895,17.0574482065323,-18.5061201348387));
#45862=CARTESIAN_POINT('Ctrl Pts',(17.2772850559938,17.104189849021,-18.5102897007821));
#45863=CARTESIAN_POINT('Ctrl Pts',(17.2097430958424,17.1542450583193,-18.5144592667256));
#45864=CARTESIAN_POINT('Ctrl Pts',(17.1398264436722,17.206060147043,-18.5187754294652));
#45865=CARTESIAN_POINT('Ctrl Pts',(17.0725797574076,17.2614258339336,-18.5230915922048));
#45866=CARTESIAN_POINT('Ctrl Pts',(17.0083685115613,17.3200224839759,-18.5274077549445));
#45867=CARTESIAN_POINT('Ctrl Pts',(16.9462489403141,17.3767103542885,-18.5315833191356));
#45868=CARTESIAN_POINT('Ctrl Pts',(16.8869703858411,17.4364215555155,-18.5357588833266));
#45869=CARTESIAN_POINT('Ctrl Pts',(16.8308254399579,17.4988298583352,-18.5399344475177));
#45870=CARTESIAN_POINT('Ctrl Pts',(16.7718447463028,17.5643902561989,-18.5443209095316));
#45871=CARTESIAN_POINT('Ctrl Pts',(16.7163229051916,17.6329269235817,-18.5487073715455));
#45872=CARTESIAN_POINT('Ctrl Pts',(16.6645491064847,17.7040252160939,-18.5530938335595));
#45873=CARTESIAN_POINT('Ctrl Pts',(16.6127753077779,17.775123508606,-18.5574802955734));
#45874=CARTESIAN_POINT('Ctrl Pts',(16.5647498046499,17.8487828986679,-18.5618667575873));
#45875=CARTESIAN_POINT('Ctrl Pts',(16.5207062260027,17.924558913131,-18.5662532196012));
#45876=CARTESIAN_POINT('Ctrl Pts',(16.4770273612299,17.9997074453442,-18.5706033584188));
#45877=CARTESIAN_POINT('Ctrl Pts',(16.4371122169921,18.0771985084612,-18.5749534972363));
#45878=CARTESIAN_POINT('Ctrl Pts',(16.4012086273385,18.1566355413635,-18.5793036360539));
#45879=CARTESIAN_POINT('Ctrl Pts',(16.3640774712899,18.2387885765663,-18.5838025088637));
#45880=CARTESIAN_POINT('Ctrl Pts',(16.3312374248385,18.3230227236652,-18.5883013816735));
#45881=CARTESIAN_POINT('Ctrl Pts',(16.3029130373493,18.4088677290933,-18.5928002544833));
#45882=CARTESIAN_POINT('Ctrl Pts',(16.2756354411695,18.4915401396801,-18.5971328613513));
#45883=CARTESIAN_POINT('Ctrl Pts',(16.2525458055772,18.5757060184788,-18.6014654682194));
#45884=CARTESIAN_POINT('Ctrl Pts',(16.2337970621827,18.660922487526,-18.6057980750875));
#45885=CARTESIAN_POINT('Ctrl Pts',(16.2150725182344,18.7460289656627,-18.6101250897576));
#45886=CARTESIAN_POINT('Ctrl Pts',(16.2006778102744,18.8321829392905,-18.6144521044276));
#45887=CARTESIAN_POINT('Ctrl Pts',(16.1907160845812,18.9189265065566,-18.6187791190976));
#45888=CARTESIAN_POINT('Ctrl Pts',(16.1807681682272,19.005549826451,-18.6231001354883));
#45889=CARTESIAN_POINT('Ctrl Pts',(16.1752410444519,19.0927607071638,-18.6274211518791));
#45890=CARTESIAN_POINT('Ctrl Pts',(16.1741865858058,19.1800923227742,-18.6317421682699));
#45891=CARTESIAN_POINT('Ctrl Pts',(16.1740606709629,19.190520751334,-18.6322581487704));
#45892=CARTESIAN_POINT('Ctrl Pts',(16.1739984722012,19.2009508929684,-18.632774129271));
#45893=CARTESIAN_POINT('Ctrl Pts',(16.1740000284928,19.2113819467091,-18.6332901097715));
#45894=CARTESIAN_POINT('Ctrl Pts',(16.1781629602604,19.2113866753936,-18.633290374834));
#45895=CARTESIAN_POINT('Ctrl Pts',(16.1776269335845,19.615981772308,-18.6533365919835));
#45896=CARTESIAN_POINT('Ctrl Pts',(16.4590846999913,20.8754715672834,-18.7157747446936));
#45897=CARTESIAN_POINT('Ctrl Pts',(18.237060364334,22.0893673291904,-18.8102032533429));
#45898=CARTESIAN_POINT('Ctrl Pts',(19.7793305876597,21.6276026831124,-18.8845855448426));
#45899=CARTESIAN_POINT('Ctrl Pts',(20.2933494018237,21.2408835667842,-18.9165759007818));
#45900=CARTESIAN_POINT('',(16.1740000028035,19.2111198080496,-18.5667098901964));
#45901=CARTESIAN_POINT('Ctrl Pts',(16.1740000028035,19.2111198086916,-18.5667098902285));
#45902=CARTESIAN_POINT('Ctrl Pts',(16.1740003013853,19.2174997239769,-18.5670291853155));
#45903=CARTESIAN_POINT('Ctrl Pts',(16.1740244495167,19.223879573923,-18.5673484804024));
#45904=CARTESIAN_POINT('Ctrl Pts',(16.1740724460423,19.2302592442234,-18.5676677754894));
#45905=CARTESIAN_POINT('Ctrl Pts',(16.1747014814392,19.31387026376,-18.5718524098819));
#45906=CARTESIAN_POINT('Ctrl Pts',(16.1794322843349,19.3976060296583,-18.5760370442745));
#45907=CARTESIAN_POINT('Ctrl Pts',(16.1882813814472,19.4810309522136,-18.580221678667));
#45908=CARTESIAN_POINT('Ctrl Pts',(16.197117882965,19.5643371297178,-18.5844003567505));
#45909=CARTESIAN_POINT('Ctrl Pts',(16.2100609870472,19.6473328891642,-18.5885790348339));
#45910=CARTESIAN_POINT('Ctrl Pts',(16.2270752140173,19.7295827970784,-18.5927577129174));
#45911=CARTESIAN_POINT('Ctrl Pts',(16.2443944087804,19.8133069754922,-18.5970112908029));
#45912=CARTESIAN_POINT('Ctrl Pts',(16.2659321081158,19.8962578184692,-18.6012648686885));
#45913=CARTESIAN_POINT('Ctrl Pts',(16.2915956147073,19.9779816286607,-18.6055184465741));
#45914=CARTESIAN_POINT('Ctrl Pts',(16.3167615841416,20.058121063309,-18.6096895605515));
#45915=CARTESIAN_POINT('Ctrl Pts',(16.3458946705845,20.1370801583406,-18.613860674529));
#45916=CARTESIAN_POINT('Ctrl Pts',(16.3788563531112,20.2144432731945,-18.6180317885065));
#45917=CARTESIAN_POINT('Ctrl Pts',(16.4118069750271,20.2917804281082,-18.6222015028263));
#45918=CARTESIAN_POINT('Ctrl Pts',(16.4485834613786,20.3675222435802,-18.6263712171462));
#45919=CARTESIAN_POINT('Ctrl Pts',(16.4889988104969,20.4412721890418,-18.6305409314661));
#45920=CARTESIAN_POINT('Ctrl Pts',(16.5294127214636,20.5150195101638,-18.6347104974097));
#45921=CARTESIAN_POINT('Ctrl Pts',(16.5734650159173,20.5867746991837,-18.6388800633532));
#45922=CARTESIAN_POINT('Ctrl Pts',(16.620922959331,20.6561662258016,-18.6430496292968));
#45923=CARTESIAN_POINT('Ctrl Pts',(16.6700494655017,20.7279974729095,-18.6473657920363));
#45924=CARTESIAN_POINT('Ctrl Pts',(16.7228252639787,20.7972953169818,-18.6516819547758));
#45925=CARTESIAN_POINT('Ctrl Pts',(16.7789448088305,20.8636824254772,-18.6559981175153));
#45926=CARTESIAN_POINT('Ctrl Pts',(16.8332362653982,20.9279069808804,-18.6601736817065));
#45927=CARTESIAN_POINT('Ctrl Pts',(16.8906566126945,20.9894072108734,-18.6643492458977));
#45928=CARTESIAN_POINT('Ctrl Pts',(16.9508909514353,21.0478783631277,-18.668524810089));
#45929=CARTESIAN_POINT('Ctrl Pts',(17.0141675834551,21.1093027543025,-18.6729112721026));
#45930=CARTESIAN_POINT('Ctrl Pts',(17.0805495076474,21.1673836440658,-18.6772977341163));
#45931=CARTESIAN_POINT('Ctrl Pts',(17.149633344248,21.2218163268039,-18.6816841961299));
#45932=CARTESIAN_POINT('Ctrl Pts',(17.2187171808487,21.276249009542,-18.6860706581435));
#45933=CARTESIAN_POINT('Ctrl Pts',(17.2905024122582,21.327033212256,-18.6904571201572));
#45934=CARTESIAN_POINT('Ctrl Pts',(17.3645537444777,21.3739186191894,-18.6948435821708));
#45935=CARTESIAN_POINT('Ctrl Pts',(17.435197865104,21.4186467590315,-18.6990282165633));
#45936=CARTESIAN_POINT('Ctrl Pts',(17.5081670866297,21.4599934843659,-18.7032128509557));
#45937=CARTESIAN_POINT('Ctrl Pts',(17.5831040926458,21.497709122393,-18.7073974853482));
#45938=CARTESIAN_POINT('Ctrl Pts',(17.6579344351091,21.5353710768775,-18.7115761634316));
#45939=CARTESIAN_POINT('Ctrl Pts',(17.7347265911908,21.5694120050826,-18.7157548415149));
#45940=CARTESIAN_POINT('Ctrl Pts',(17.8130952257718,21.5996260479204,-18.7199335195983));
#45941=CARTESIAN_POINT('Ctrl Pts',(17.8928685618191,21.630381655767,-18.7241870974839));
#45942=CARTESIAN_POINT('Ctrl Pts',(17.9742750416618,21.6571715770568,-18.7284406753695));
#45943=CARTESIAN_POINT('Ctrl Pts',(18.0568830023299,21.6798281777933,-18.732694253255));
#45944=CARTESIAN_POINT('Ctrl Pts',(18.1378894464698,21.7020455361098,-18.7368653672324));
#45945=CARTESIAN_POINT('Ctrl Pts',(18.2200507369794,21.7202882813848,-18.7410364812097));
#45946=CARTESIAN_POINT('Ctrl Pts',(18.3029424071742,21.734447909442,-18.7452075951871));
#45947=CARTESIAN_POINT('Ctrl Pts',(18.3858062622684,21.7486027860993,-18.7493773095069));
#45948=CARTESIAN_POINT('Ctrl Pts',(18.469399557216,21.7586771892408,-18.7535470238266));
#45949=CARTESIAN_POINT('Ctrl Pts',(18.5532876521045,21.7646137232005,-18.7577167381464));
#45950=CARTESIAN_POINT('Ctrl Pts',(18.6371727618945,21.7705500459129,-18.7618863040899));
#45951=CARTESIAN_POINT('Ctrl Pts',(18.7213521918226,21.7723487605766,-18.7660558700333));
#45952=CARTESIAN_POINT('Ctrl Pts',(18.8053875689174,21.7700044577929,-18.7702254359767));
#45953=CARTESIAN_POINT('Ctrl Pts',(18.8923775262288,21.7675777322146,-18.7745415987164));
#45954=CARTESIAN_POINT('Ctrl Pts',(18.9792125852182,21.7607112463061,-18.778857761456));
#45955=CARTESIAN_POINT('Ctrl Pts',(19.0654100827151,21.7494576728941,-18.7831739241956));
#45956=CARTESIAN_POINT('Ctrl Pts',(19.1487997057715,21.7385706834556,-18.7873494883867));
#45957=CARTESIAN_POINT('Ctrl Pts',(19.2315922114994,21.7235781663988,-18.7915250525778));
#45958=CARTESIAN_POINT('Ctrl Pts',(19.3133609024084,21.7045799455322,-18.7957006167688));
#45959=CARTESIAN_POINT('Ctrl Pts',(19.3992595355479,21.6846221696845,-18.8000870787827));
#45960=CARTESIAN_POINT('Ctrl Pts',(19.4840276488775,21.6602435606427,-18.8044735407967));
#45961=CARTESIAN_POINT('Ctrl Pts',(19.5671906913808,21.6316183655827,-18.8088600028106));
#45962=CARTESIAN_POINT('Ctrl Pts',(19.6503537338841,21.6029931705227,-18.8132464648245));
#45963=CARTESIAN_POINT('Ctrl Pts',(19.7319111958455,21.5701216768946,-18.8176329268384));
#45964=CARTESIAN_POINT('Ctrl Pts',(19.8114169849415,21.5332344068934,-18.8220193888523));
#45965=CARTESIAN_POINT('Ctrl Pts',(19.8872706217464,21.4980415786326,-18.8262043557616));
#45966=CARTESIAN_POINT('Ctrl Pts',(19.9615393050008,21.4590628106808,-18.8303893226708));
#45967=CARTESIAN_POINT('Ctrl Pts',(20.0338195953317,21.4164634478022,-18.8345742895801));
#45968=CARTESIAN_POINT('Ctrl Pts',(20.1059885648699,21.3739296933326,-18.8387528111108));
#45969=CARTESIAN_POINT('Ctrl Pts',(20.1761748342838,21.327786657028,-18.8429313326415));
#45970=CARTESIAN_POINT('Ctrl Pts',(20.2439967783601,21.2782468960775,-18.8471098541722));
#45971=CARTESIAN_POINT('Ctrl Pts',(20.2606541302848,21.2660797244687,-18.8481361164625));
#45972=CARTESIAN_POINT('Ctrl Pts',(20.2771689741761,21.2537078773064,-18.8491623787528));
#45973=CARTESIAN_POINT('Ctrl Pts',(20.2935358855687,21.2411349269503,-18.8501886410431));
#45974=CARTESIAN_POINT('Ctrl Pts',(20.2935358855687,21.2411349269503,-18.0500683201495));
#45975=CARTESIAN_POINT('Ctrl Pts',(20.3406388660272,21.2049507367435,-18.0530337296876));
#45976=CARTESIAN_POINT('Ctrl Pts',(20.3864285990884,21.1671673046285,-18.0559991392257));
#45977=CARTESIAN_POINT('Ctrl Pts',(20.4307957154104,21.1278944415812,-18.0589645487637));
#45978=CARTESIAN_POINT('Ctrl Pts',(20.4934043225861,21.0724745842854,-18.0631491831568));
#45979=CARTESIAN_POINT('Ctrl Pts',(20.5534114448285,21.0138810328615,-18.0673338175499));
#45980=CARTESIAN_POINT('Ctrl Pts',(20.6104778947951,20.9523875818856,-18.071518451943));
#45981=CARTESIAN_POINT('Ctrl Pts',(20.6674631177336,20.8909816592258,-18.0756971300271));
#45982=CARTESIAN_POINT('Ctrl Pts',(20.7215156722283,20.8266843701416,-18.0798758081111));
#45983=CARTESIAN_POINT('Ctrl Pts',(20.7723306651573,20.7598086064712,-18.0840544861951));
#45984=CARTESIAN_POINT('Ctrl Pts',(20.8240564803136,20.691734142801,-18.0883080640805));
#45985=CARTESIAN_POINT('Ctrl Pts',(20.8724271646772,20.620988176579,-18.0925616419659));
#45986=CARTESIAN_POINT('Ctrl Pts',(20.91716165977,20.5479387298267,-18.0968152198513));
#45987=CARTESIAN_POINT('Ctrl Pts',(20.9610288893839,20.4763054891426,-18.1009863338293));
#45988=CARTESIAN_POINT('Ctrl Pts',(21.0013994094997,20.4024576962096,-18.1051574478073));
#45989=CARTESIAN_POINT('Ctrl Pts',(21.0380509604127,20.326772903337,-18.1093285617853));
#45990=CARTESIAN_POINT('Ctrl Pts',(21.0746902125439,20.2511135072277,-18.1134982761058));
#45991=CARTESIAN_POINT('Ctrl Pts',(21.1076127735552,20.1736187490991,-18.1176679904262));
#45992=CARTESIAN_POINT('Ctrl Pts',(21.136642647489,20.0946901654241,-18.1218377047466));
#45993=CARTESIAN_POINT('Ctrl Pts',(21.1656714884152,20.0157643903668,-18.1260072706907));
#45994=CARTESIAN_POINT('Ctrl Pts',(21.1908077596747,19.9354053232572,-18.1301768366348));
#45995=CARTESIAN_POINT('Ctrl Pts',(21.211924363067,19.8540325426593,-18.1343464025789));
#45996=CARTESIAN_POINT('Ctrl Pts',(21.2337834001838,19.7697987954824,-18.1386625653178));
#45997=CARTESIAN_POINT('Ctrl Pts',(21.2513347146947,19.6844792346864,-18.1429787280566));
#45998=CARTESIAN_POINT('Ctrl Pts',(21.2644946836059,19.5985521335796,-18.1472948907955));
#45999=CARTESIAN_POINT('Ctrl Pts',(21.2772259679144,19.5154240987509,-18.1514704549872));
#46000=CARTESIAN_POINT('Ctrl Pts',(21.2858476079666,19.4317279704215,-18.1556460191789));
#46001=CARTESIAN_POINT('Ctrl Pts',(21.290336834896,19.3479013752814,-18.1598215833707));
#46002=CARTESIAN_POINT('Ctrl Pts',(21.2950528020053,19.2598408981036,-18.1642080453831));
#46003=CARTESIAN_POINT('Ctrl Pts',(21.295207927637,19.1716370118692,-18.1685945073955));
#46004=CARTESIAN_POINT('Ctrl Pts',(21.2908376238657,19.083794004918,-18.1729809694079));
#46005=CARTESIAN_POINT('Ctrl Pts',(21.2864673200944,18.9959509979668,-18.1773674314203));
#46006=CARTESIAN_POINT('Ctrl Pts',(21.2775717212916,18.9084694398441,-18.1817538934327));
#46007=CARTESIAN_POINT('Ctrl Pts',(21.2642482087237,18.8218419315364,-18.1861403554451));
#46008=CARTESIAN_POINT('Ctrl Pts',(21.251537730719,18.7392002832971,-18.1903249898381));
#46009=CARTESIAN_POINT('Ctrl Pts',(21.2347505437474,18.6570282117551,-18.194509624231));
#46010=CARTESIAN_POINT('Ctrl Pts',(21.2139332700432,18.5757591195989,-18.198694258624));
#46011=CARTESIAN_POINT('Ctrl Pts',(21.1931456271515,18.4946057039364,-18.2028729367079));
#46012=CARTESIAN_POINT('Ctrl Pts',(21.1683394048595,18.4143531565236,-18.2070516147918));
#46013=CARTESIAN_POINT('Ctrl Pts',(21.1396126628228,18.3354272066433,-18.2112302928757));
#46014=CARTESIAN_POINT('Ctrl Pts',(21.1103710145802,18.2550865658331,-18.2154838707611));
#46015=CARTESIAN_POINT('Ctrl Pts',(21.0770669868029,18.1761210253964,-18.2197374486466));
#46016=CARTESIAN_POINT('Ctrl Pts',(21.0398578961466,18.098966114375,-18.223991026532));
#46017=CARTESIAN_POINT('Ctrl Pts',(21.0033701763209,18.0233070018604,-18.2281621405099));
#46018=CARTESIAN_POINT('Ctrl Pts',(20.9631276659834,17.9493893735374,-18.2323332544878));
#46019=CARTESIAN_POINT('Ctrl Pts',(20.9193275219149,17.8776044765482,-18.2365043684657));
#46020=CARTESIAN_POINT('Ctrl Pts',(20.8755420754078,17.8058436676746,-18.2406740827861));
#46021=CARTESIAN_POINT('Ctrl Pts',(20.8282016054844,17.7362145612029,-18.2448437971064));
#46022=CARTESIAN_POINT('Ctrl Pts',(20.7775484775,17.6690824859586,-18.2490135114267));
#46023=CARTESIAN_POINT('Ctrl Pts',(20.7268971519712,17.6019527995616,-18.2531830773707));
#46024=CARTESIAN_POINT('Ctrl Pts',(20.6729336805178,17.5373203344384,-18.2573526433147));
#46025=CARTESIAN_POINT('Ctrl Pts',(20.6159420664671,17.4755190699804,-18.2615222092586));
#46026=CARTESIAN_POINT('Ctrl Pts',(20.5569466975713,17.4115449493023,-18.2658383719976));
#46027=CARTESIAN_POINT('Ctrl Pts',(20.4947066427113,17.3506052113062,-18.2701545347366));
#46028=CARTESIAN_POINT('Ctrl Pts',(20.4295787905104,17.2930290499668,-18.2744706974756));
#46029=CARTESIAN_POINT('Ctrl Pts',(20.3665724712465,17.2373284260287,-18.2786462616672));
#46030=CARTESIAN_POINT('Ctrl Pts',(20.300864002761,17.1847758643075,-18.2828218258589));
#46031=CARTESIAN_POINT('Ctrl Pts',(20.2328090354887,17.1356273888438,-18.2869973900505));
#46032=CARTESIAN_POINT('Ctrl Pts',(20.1613167736019,17.0839965407216,-18.2913838520632));
#46033=CARTESIAN_POINT('Ctrl Pts',(20.0872352304045,17.0361230139113,-18.2957703140758));
#46034=CARTESIAN_POINT('Ctrl Pts',(20.0110076004693,16.9922499941761,-18.3001567760885));
#46035=CARTESIAN_POINT('Ctrl Pts',(19.9347799705342,16.9483769744409,-18.3045432381012));
#46036=CARTESIAN_POINT('Ctrl Pts',(19.8564068054917,16.9085046570797,-18.3089297001138));
#46037=CARTESIAN_POINT('Ctrl Pts',(19.7763550154481,16.8728177954295,-18.3133161621265));
#46038=CARTESIAN_POINT('Ctrl Pts',(19.6999865269337,16.8387729391862,-18.3175007965194));
#46039=CARTESIAN_POINT('Ctrl Pts',(19.6218062328668,16.8084101229908,-18.3216854309124));
#46040=CARTESIAN_POINT('Ctrl Pts',(19.5422037920521,16.7819247375776,-18.3258700653053));
#46041=CARTESIAN_POINT('Ctrl Pts',(19.4627146554591,16.7554770508322,-18.3300487433892));
#46042=CARTESIAN_POINT('Ctrl Pts',(19.3818078256876,16.7328959763056,-18.334227421473));
#46043=CARTESIAN_POINT('Ctrl Pts',(19.2998943515232,16.7143295005319,-18.3384060995568));
#46044=CARTESIAN_POINT('Ctrl Pts',(19.2165126372019,16.6954302340229,-18.3426596774423));
#46045=CARTESIAN_POINT('Ctrl Pts',(19.1320882756871,16.6806911015683,-18.3469132553277));
#46046=CARTESIAN_POINT('Ctrl Pts',(19.0470726305013,16.6702155683665,-18.3511668332132));
#46047=CARTESIAN_POINT('Ctrl Pts',(18.9637051794946,16.6599431238176,-18.3553379471911));
#46048=CARTESIAN_POINT('Ctrl Pts',(18.8797696442083,16.6537704962434,-18.3595090611689));
#46049=CARTESIAN_POINT('Ctrl Pts',(18.795701718799,16.6517436826497,-18.3636801751467));
#46050=CARTESIAN_POINT('Ctrl Pts',(18.711662003194,16.649717549173,-18.367849889467));
#46051=CARTESIAN_POINT('Ctrl Pts',(18.6274904452109,16.6518344778738,-18.3720196037873));
#46052=CARTESIAN_POINT('Ctrl Pts',(18.5436254163474,16.6580884234077,-18.3761893181075));
#46053=CARTESIAN_POINT('Ctrl Pts',(18.4597633717615,16.6643421463994,-18.3803588840515));
#46054=CARTESIAN_POINT('Ctrl Pts',(18.3762082933037,16.6747325584671,-18.3845284499954));
#46055=CARTESIAN_POINT('Ctrl Pts',(18.2933947304034,16.6892016344672,-18.3886980159393));
#46056=CARTESIAN_POINT('Ctrl Pts',(18.2076695447882,16.7041794253309,-18.3930141786784));
#46057=CARTESIAN_POINT('Ctrl Pts',(18.122739507835,16.7235279374021,-18.3973303414174));
#46058=CARTESIAN_POINT('Ctrl Pts',(18.0390745966233,16.7471252702823,-18.4016465041565));
#46059=CARTESIAN_POINT('Ctrl Pts',(17.958135061099,16.7699539225246,-18.405822068348));
#46060=CARTESIAN_POINT('Ctrl Pts',(17.8783799255841,16.7967586410081,-18.4099976325396));
#46061=CARTESIAN_POINT('Ctrl Pts',(17.8002169726149,16.8273789609572,-18.4141731967312));
#46062=CARTESIAN_POINT('Ctrl Pts',(17.7181061946991,16.8595458404768,-18.418559658744));
#46063=CARTESIAN_POINT('Ctrl Pts',(17.6377532005338,16.895923662579,-18.4229461207568));
#46064=CARTESIAN_POINT('Ctrl Pts',(17.5596023636775,16.9362714026064,-18.4273325827696));
#46065=CARTESIAN_POINT('Ctrl Pts',(17.4814515268212,16.9766191426339,-18.4317190447824));
#46066=CARTESIAN_POINT('Ctrl Pts',(17.4055033100763,17.0209364424643,-18.4361055067952));
#46067=CARTESIAN_POINT('Ctrl Pts',(17.3321657913463,17.0689307080656,-18.4404919688079));
#46068=CARTESIAN_POINT('Ctrl Pts',(17.2622960528831,17.1146555545476,-18.4446710160258));
#46069=CARTESIAN_POINT('Ctrl Pts',(17.19453408493,17.1638887348098,-18.4488500632436));
#46070=CARTESIAN_POINT('Ctrl Pts',(17.1292545139166,17.2164093339998,-18.4530291104615));
#46071=CARTESIAN_POINT('Ctrl Pts',(17.0640679209106,17.2688551278475,-18.4572022054423));
#46072=CARTESIAN_POINT('Ctrl Pts',(17.0013570587502,17.3245787540421,-18.461375300423));
#46073=CARTESIAN_POINT('Ctrl Pts',(16.9414683281886,17.3833156165374,-18.4655483954038));
#46074=CARTESIAN_POINT('Ctrl Pts',(16.8809773183909,17.4426431743496,-18.4697634576868));
#46075=CARTESIAN_POINT('Ctrl Pts',(16.8233659292104,17.5050446643084,-18.4739785199699));
#46076=CARTESIAN_POINT('Ctrl Pts',(16.7689574885197,17.5702050926227,-18.4781935822529));
#46077=CARTESIAN_POINT('Ctrl Pts',(16.7151877112471,17.6346006473008,-18.4823591668069));
#46078=CARTESIAN_POINT('Ctrl Pts',(16.6645463875622,17.701690347722,-18.4865247513609));
#46079=CARTESIAN_POINT('Ctrl Pts',(16.6173078768048,17.7711338758054,-18.4906903359149));
#46080=CARTESIAN_POINT('Ctrl Pts',(16.5700850499658,17.84055434756,-18.4948545374302));
#46081=CARTESIAN_POINT('Ctrl Pts',(16.5262630517187,17.9123267137652,-18.4990187389455));
#46082=CARTESIAN_POINT('Ctrl Pts',(16.4860739671285,17.9860801859963,-18.5031829404608));
#46083=CARTESIAN_POINT('Ctrl Pts',(16.4458860826637,18.0598314558034,-18.5073470176248));
#46084=CARTESIAN_POINT('Ctrl Pts',(16.4093311160891,18.1355633083681,-18.5115110947889));
#46085=CARTESIAN_POINT('Ctrl Pts',(16.3765953977375,18.2128799965778,-18.5156751719529));
#46086=CARTESIAN_POINT('Ctrl Pts',(16.3431614559388,18.2918457802489,-18.5199280651398));
#46087=CARTESIAN_POINT('Ctrl Pts',(16.3137117771032,18.3724643312945,-18.5241809583268));
#46088=CARTESIAN_POINT('Ctrl Pts',(16.2883925214927,18.4542939401133,-18.5284338515138));
#46089=CARTESIAN_POINT('Ctrl Pts',(16.2635663208298,18.534530038676,-18.5326039259141));
#46090=CARTESIAN_POINT('Ctrl Pts',(16.2427111716314,18.6159299801766,-18.5367740003144));
#46091=CARTESIAN_POINT('Ctrl Pts',(16.2259135016088,18.6980651926532,-18.5409440747148));
#46092=CARTESIAN_POINT('Ctrl Pts',(16.2086154222953,18.7826472458752,-18.545238377295));
#46093=CARTESIAN_POINT('Ctrl Pts',(16.1956204803926,18.8680085473305,-18.5495326798753));
#46094=CARTESIAN_POINT('Ctrl Pts',(16.1869656326132,18.9536754357807,-18.5538269824556));
#46095=CARTESIAN_POINT('Ctrl Pts',(16.1783107848339,19.0393423242308,-18.5581212850358));
#46096=CARTESIAN_POINT('Ctrl Pts',(16.1739959871027,19.125314270194,-18.5624155876161));
#46097=CARTESIAN_POINT('Ctrl Pts',(16.1740000028035,19.2111198080496,-18.5667098901964));
#46098=CARTESIAN_POINT('Origin',(18.734,19.211,1.76670989022852));
#46099=CARTESIAN_POINT('',(20.2917780654113,21.2388105542775,-17.2500265414872));
#46100=CARTESIAN_POINT('',(20.2944552762682,21.2423103685662,-17.3168007019908));
#46101=CARTESIAN_POINT('',(20.2935358855687,21.2411349269503,1.76670989022852));
#46102=CARTESIAN_POINT('',(16.1740010840393,19.2086440968075,-17.8332901097715));
#46103=CARTESIAN_POINT('Ctrl Pts',(20.2944552762683,21.2423103685662,-17.3168007019908));
#46104=CARTESIAN_POINT('Ctrl Pts',(20.8466207046277,20.8094281841944,-17.3517574544833));
#46105=CARTESIAN_POINT('Ctrl Pts',(21.6812137731847,19.3312716956158,-17.4291061425363));
#46106=CARTESIAN_POINT('Ctrl Pts',(20.5976437728566,16.8256022375524,-17.5488467661498));
#46107=CARTESIAN_POINT('Ctrl Pts',(17.7370130066076,16.3527999488813,-17.6760225728312));
#46108=CARTESIAN_POINT('Ctrl Pts',(16.286227466659,17.9552740380232,-17.7708370079901));
#46109=CARTESIAN_POINT('Ctrl Pts',(16.1722336618266,19.0070072559387,-17.8232595075886));
#46110=CARTESIAN_POINT('Ctrl Pts',(16.1740883584118,19.2086434103328,-17.8332900716265));
#46111=CARTESIAN_POINT('Ctrl Pts',(16.1740010840393,19.2086440968075,-17.8332901097715));
#46112=CARTESIAN_POINT('Ctrl Pts',(16.1739248258781,19.2915086264566,-17.837412174938));
#46113=CARTESIAN_POINT('Ctrl Pts',(16.177876160498,19.3744847533445,-17.8415342401044));
#46114=CARTESIAN_POINT('Ctrl Pts',(16.1858608731257,19.4571442465142,-17.8456563052709));
#46115=CARTESIAN_POINT('Ctrl Pts',(16.1938402258665,19.5397482529614,-17.8497756034244));
#46116=CARTESIAN_POINT('Ctrl Pts',(16.205847540348,19.6220355783689,-17.853894901578));
#46117=CARTESIAN_POINT('Ctrl Pts',(16.2218365582967,19.7035797825425,-17.8580141997315));
#46118=CARTESIAN_POINT('Ctrl Pts',(16.2378199266111,19.7850951735058,-17.862132042353));
#46119=CARTESIAN_POINT('Ctrl Pts',(16.2577821151893,19.8658675009388,-17.8662498849745));
#46120=CARTESIAN_POINT('Ctrl Pts',(16.2816254461127,19.9454787590162,-17.8703677275959));
#46121=CARTESIAN_POINT('Ctrl Pts',(16.3054679320359,20.0250871956956,-17.8744854242824));
#46122=CARTESIAN_POINT('Ctrl Pts',(16.3331911499574,20.1035341923719,-17.8786031209688));
#46123=CARTESIAN_POINT('Ctrl Pts',(16.364647494651,20.1804166830608,-17.8827208176552));
#46124=CARTESIAN_POINT('Ctrl Pts',(16.396133878009,20.257372591286,-17.8868424464612));
#46125=CARTESIAN_POINT('Ctrl Pts',(16.4313603282317,20.3327605713697,-17.8909640752672));
#46126=CARTESIAN_POINT('Ctrl Pts',(16.4701312380089,20.4061979871474,-17.8950857040732));
#46127=CARTESIAN_POINT('Ctrl Pts',(16.5089205032735,20.479670170733,-17.8992092842006));
#46128=CARTESIAN_POINT('Ctrl Pts',(16.5512573267502,20.5511895451374,-17.903332864328));
#46129=CARTESIAN_POINT('Ctrl Pts',(16.5969016205558,20.6204007650689,-17.9074564444553));
#46130=CARTESIAN_POINT('Ctrl Pts',(16.6426258760309,20.6897332322415,-17.9115872484507));
#46131=CARTESIAN_POINT('Ctrl Pts',(16.6916688941171,20.7567490876318,-17.915718052446));
#46132=CARTESIAN_POINT('Ctrl Pts',(16.743749207993,20.8211247730892,-17.9198488564413));
#46133=CARTESIAN_POINT('Ctrl Pts',(16.7879829276106,20.8758014024869,-17.9233572996922));
#46134=CARTESIAN_POINT('Ctrl Pts',(16.8344068718463,20.9285739549632,-17.9268657429432));
#46135=CARTESIAN_POINT('Ctrl Pts',(16.8828286089276,20.979265953095,-17.9303741861941));
#46136=CARTESIAN_POINT('Ctrl Pts',(16.9405827898753,21.039727948248,-17.9345588205871));
#46137=CARTESIAN_POINT('Ctrl Pts',(17.0014097311532,21.0974699797563,-17.9387434549801));
#46138=CARTESIAN_POINT('Ctrl Pts',(17.0650229727701,21.152163486824,-17.9429280893731));
#46139=CARTESIAN_POINT('Ctrl Pts',(17.1285456688113,21.2067791444541,-17.947106767457));
#46140=CARTESIAN_POINT('Ctrl Pts',(17.1948464417153,21.2583545993042,-17.9512854455409));
#46141=CARTESIAN_POINT('Ctrl Pts',(17.2636010628233,21.3065970427421,-17.9554641236248));
#46142=CARTESIAN_POINT('Ctrl Pts',(17.3335880611026,21.3557041973082,-17.9597177015102));
#46143=CARTESIAN_POINT('Ctrl Pts',(17.4061174102899,21.4013573280785,-17.9639712793957));
#46144=CARTESIAN_POINT('Ctrl Pts',(17.4808106950311,21.4432895345164,-17.9682248572811));
#46145=CARTESIAN_POINT('Ctrl Pts',(17.5540559046944,21.4844088033079,-17.972395971259));
#46146=CARTESIAN_POINT('Ctrl Pts',(17.6293814748144,21.5219498994727,-17.9765670852369));
#46147=CARTESIAN_POINT('Ctrl Pts',(17.7064016963161,21.555705040355,-17.9807381992148));
#46148=CARTESIAN_POINT('Ctrl Pts',(17.7833960729386,21.5894488543737,-17.9849079135351));
#46149=CARTESIAN_POINT('Ctrl Pts',(17.8620835505881,21.6194090516659,-17.9890776278554));
#46150=CARTESIAN_POINT('Ctrl Pts',(17.9420562076474,21.6454249895518,-17.9932473421757));
#46151=CARTESIAN_POINT('Ctrl Pts',(18.0220260189365,21.671440001679,-17.9974169081197));
#46152=CARTESIAN_POINT('Ctrl Pts',(18.1032804809775,21.6935108919569,-18.0015864740637));
#46153=CARTESIAN_POINT('Ctrl Pts',(18.1853954972943,21.7115265644682,-18.0057560400077));
#46154=CARTESIAN_POINT('Ctrl Pts',(18.2703975762873,21.7301756458007,-18.0100722027467));
#46155=CARTESIAN_POINT('Ctrl Pts',(18.3563213344854,21.7444789277004,-18.0143883654857));
#46156=CARTESIAN_POINT('Ctrl Pts',(18.4426856715115,21.7543709839536,-18.0187045282247));
#46157=CARTESIAN_POINT('Ctrl Pts',(18.5262366993405,21.7639408075146,-18.0228800924163));
#46158=CARTESIAN_POINT('Ctrl Pts',(18.6101995699749,21.7693824000208,-18.0270556566079));
#46159=CARTESIAN_POINT('Ctrl Pts',(18.6941361080732,21.7706896042529,-18.0312312207995));
#46160=CARTESIAN_POINT('Ctrl Pts',(18.7823120811743,21.7720628322632,-18.0356176828122));
#46161=CARTESIAN_POINT('Ctrl Pts',(18.870458408217,21.7688730610124,-18.0400041448249));
#46162=CARTESIAN_POINT('Ctrl Pts',(18.9580725064404,21.7611748002554,-18.0443906068375));
#46163=CARTESIAN_POINT('Ctrl Pts',(19.0456866046639,21.7534765394983,-18.0487770688502));
#46164=CARTESIAN_POINT('Ctrl Pts',(19.132767910028,21.7412699451077,-18.0531635308629));
#46165=CARTESIAN_POINT('Ctrl Pts',(19.2188278686568,21.7246710082614,-18.0575499928755));
#46166=CARTESIAN_POINT('Ctrl Pts',(19.3009320014004,21.7088350569554,-18.06173482709));
#46167=CARTESIAN_POINT('Ctrl Pts',(19.3824122424305,21.6889427479766,-18.0659196613044));
#46168=CARTESIAN_POINT('Ctrl Pts',(19.4628372070827,21.665057115385,-18.0701044955188));
#46169=CARTESIAN_POINT('Ctrl Pts',(19.5431287709647,21.641211101857,-18.0742823883549));
#46170=CARTESIAN_POINT('Ctrl Pts',(19.6223681012689,21.6133850633112,-18.078460281191));
#46171=CARTESIAN_POINT('Ctrl Pts',(19.7001337305628,21.5816930663139,-18.0826381740271));
#46172=CARTESIAN_POINT('Ctrl Pts',(19.7778242916652,21.5500316620208,-18.0868120338879));
#46173=CARTESIAN_POINT('Ctrl Pts',(19.8540435523394,21.5145118803042,-18.0909858937488));
#46174=CARTESIAN_POINT('Ctrl Pts',(19.928385767927,21.4752973827158,-18.0951597536096));
#46175=CARTESIAN_POINT('Ctrl Pts',(20.0026788000519,21.4361088287284,-18.0993308521204));
#46176=CARTESIAN_POINT('Ctrl Pts',(20.0750968472972,21.3932306267545,-18.1035019506312));
#46177=CARTESIAN_POINT('Ctrl Pts',(20.145255958728,21.3468737366602,-18.1076730491419));
#46178=CARTESIAN_POINT('Ctrl Pts',(20.1959047149762,21.3134081071941,-18.1106842182895));
#46179=CARTESIAN_POINT('Ctrl Pts',(20.2453766303622,21.2781305402564,-18.113695387437));
#46180=CARTESIAN_POINT('Ctrl Pts',(20.2935358855687,21.2411349269503,-18.1167065565846));
#46181=CARTESIAN_POINT('',(16.1740009581142,19.2132148462219,-17.7667099127475));
#46182=CARTESIAN_POINT('Ctrl Pts',(16.1740009581142,19.2132148462218,-17.7667099127475));
#46183=CARTESIAN_POINT('Ctrl Pts',(16.1740887027227,19.3146332252549,-17.7717442924629));
#46184=CARTESIAN_POINT('Ctrl Pts',(16.1802070184511,19.4157876786429,-17.7767786721782));
#46185=CARTESIAN_POINT('Ctrl Pts',(16.1922394471755,19.5160463769745,-17.7818130518935));
#46186=CARTESIAN_POINT('Ctrl Pts',(16.2044426849033,19.6177283198346,-17.7869188982596));
#46187=CARTESIAN_POINT('Ctrl Pts',(16.2227290670649,19.71848890314,-17.7920247446257));
#46188=CARTESIAN_POINT('Ctrl Pts',(16.2469282568518,19.8176911441861,-17.7971305909918));
#46189=CARTESIAN_POINT('Ctrl Pts',(16.2587491290717,19.8661496680319,-17.7996247057948));
#46190=CARTESIAN_POINT('Ctrl Pts',(16.2719801580739,19.9142366801005,-17.8021188205978));
#46191=CARTESIAN_POINT('Ctrl Pts',(16.2865973915759,19.9618797988219,-17.8046129354008));
#46192=CARTESIAN_POINT('Ctrl Pts',(16.3111222362101,20.0418155872439,-17.8087975697939));
#46193=CARTESIAN_POINT('Ctrl Pts',(16.3396130703746,20.1206973427815,-17.8129822041869));
#46194=CARTESIAN_POINT('Ctrl Pts',(16.3719611025222,20.1981029565358,-17.8171668385799));
#46195=CARTESIAN_POINT('Ctrl Pts',(16.4042630912499,20.2753983929799,-17.8213455166639));
#46196=CARTESIAN_POINT('Ctrl Pts',(16.440411196743,20.351221440268,-17.8255241947478));
#46197=CARTESIAN_POINT('Ctrl Pts',(16.480246839823,20.4251650188471,-17.8297028728317));
#46198=CARTESIAN_POINT('Ctrl Pts',(16.5207965081758,20.5004339829301,-17.8339564507172));
#46199=CARTESIAN_POINT('Ctrl Pts',(16.5651670712162,20.5737549756816,-17.8382100286026));
#46200=CARTESIAN_POINT('Ctrl Pts',(16.6131398985284,20.6447197878197,-17.8424636064881));
#46201=CARTESIAN_POINT('Ctrl Pts',(16.6601826789718,20.7143088085979,-17.846634720466));
#46202=CARTESIAN_POINT('Ctrl Pts',(16.7106890267626,20.7816317931436,-17.8508058344439));
#46203=CARTESIAN_POINT('Ctrl Pts',(16.7644072919754,20.8463301087231,-17.8549769484219));
#46204=CARTESIAN_POINT('Ctrl Pts',(16.8181075315056,20.911006714158,-17.8591466627423));
#46205=CARTESIAN_POINT('Ctrl Pts',(16.8750172543249,20.9730600461346,-17.8633163770626));
#46206=CARTESIAN_POINT('Ctrl Pts',(16.9348438240379,21.032163653958,-17.867486091383));
#46207=CARTESIAN_POINT('Ctrl Pts',(16.9946682648648,21.0912651586214,-17.871655657327));
#46208=CARTESIAN_POINT('Ctrl Pts',(17.0574090183537,21.1474168251239,-17.8758252232711));
#46209=CARTESIAN_POINT('Ctrl Pts',(17.1227367799309,21.2003292426475,-17.8799947892151));
#46210=CARTESIAN_POINT('Ctrl Pts',(17.1903613850148,21.2551019954968,-17.884310951954));
#46211=CARTESIAN_POINT('Ctrl Pts',(17.2607578915088,21.3064031452813,-17.888627114693));
#46212=CARTESIAN_POINT('Ctrl Pts',(17.3335255671369,21.3539585537049,-17.8929432774319));
#46213=CARTESIAN_POINT('Ctrl Pts',(17.4039228433852,21.3999648497008,-17.8971188416236));
#46214=CARTESIAN_POINT('Ctrl Pts',(17.4765387490621,21.4424654946023,-17.9012944058152));
#46215=CARTESIAN_POINT('Ctrl Pts',(17.5509843556047,21.4812585723032,-17.9054699700069));
#46216=CARTESIAN_POINT('Ctrl Pts',(17.6291900327564,21.522010996137,-17.9098564320195));
#46217=CARTESIAN_POINT('Ctrl Pts',(17.7094145736835,21.558671228602,-17.914242894032));
#46218=CARTESIAN_POINT('Ctrl Pts',(17.7911842815276,21.5910627136698,-17.9186293560446));
#46219=CARTESIAN_POINT('Ctrl Pts',(17.8729539893717,21.6234541987376,-17.9230158180571));
#46220=CARTESIAN_POINT('Ctrl Pts',(17.9562682900626,21.6515768229132,-17.9274022800697));
#46221=CARTESIAN_POINT('Ctrl Pts',(18.0406384682269,21.6753152773656,-17.9317887420822));
#46222=CARTESIAN_POINT('Ctrl Pts',(18.1211305077813,21.697962575929,-17.9359735770737));
#46223=CARTESIAN_POINT('Ctrl Pts',(18.2028831083919,21.7167042021064,-17.9401584120652));
#46224=CARTESIAN_POINT('Ctrl Pts',(18.285482396511,21.7314031342943,-17.9443432470566));
#46225=CARTESIAN_POINT('Ctrl Pts',(18.3679630513101,21.7460809551243,-17.9485220715741));
#46226=CARTESIAN_POINT('Ctrl Pts',(18.4512875288659,21.756727535889,-17.9527008960917));
#46227=CARTESIAN_POINT('Ctrl Pts',(18.5350276579567,21.7632558663076,-17.9568797206092));
#46228=CARTESIAN_POINT('Ctrl Pts',(18.6186666109275,21.7697763090965,-17.9610534962063));
#46229=CARTESIAN_POINT('Ctrl Pts',(18.7027197607572,21.7721883584651,-17.9652272718034));
#46230=CARTESIAN_POINT('Ctrl Pts',(18.7867510727816,21.7704564509521,-17.9694010474004));
#46231=CARTESIAN_POINT('Ctrl Pts',(18.8707269523644,21.7687256859164,-17.9735720697075));
#46232=CARTESIAN_POINT('Ctrl Pts',(18.9546805641743,21.7628564016082,-17.9777430920145));
#46233=CARTESIAN_POINT('Ctrl Pts',(19.0381741527011,21.7528650799813,-17.9819141143216));
#46234=CARTESIAN_POINT('Ctrl Pts',(19.1216377101411,21.7428773520466,-17.9860836363897));
#46235=CARTESIAN_POINT('Ctrl Pts',(19.2046411167496,21.7287705870409,-17.9902531584578));
#46236=CARTESIAN_POINT('Ctrl Pts',(19.2867513915052,21.7106131499072,-17.9944226805259));
#46237=CARTESIAN_POINT('Ctrl Pts',(19.3688567634635,21.6924567969525,-17.9985919536323));
#46238=CARTESIAN_POINT('Ctrl Pts',(19.4500686609559,21.6702503538458,-18.0027612267386));
#46239=CARTESIAN_POINT('Ctrl Pts',(19.5299652993015,21.6441130763505,-18.0069304998449));
#46240=CARTESIAN_POINT('Ctrl Pts',(19.6099224331149,21.6179560084503,-18.0111029298065));
#46241=CARTESIAN_POINT('Ctrl Pts',(19.6885618814567,21.5878623064593,-18.0152753597681));
#46242=CARTESIAN_POINT('Ctrl Pts',(19.7654786756144,21.5540005850944,-18.0194477897297));
#46243=CARTESIAN_POINT('Ctrl Pts',(19.84242841653,21.5201243593037,-18.0236220069219));
#46244=CARTESIAN_POINT('Ctrl Pts',(19.9176536212634,21.4824771037163,-18.027796224114));
#46245=CARTESIAN_POINT('Ctrl Pts',(19.9907728936446,21.4412739503927,-18.0319704413061));
#46246=CARTESIAN_POINT('Ctrl Pts',(20.0639908538862,21.4000151858614,-18.0361502923694));
#46247=CARTESIAN_POINT('Ctrl Pts',(20.1350968176442,21.3551911864424,-18.0403301434327));
#46248=CARTESIAN_POINT('Ctrl Pts',(20.2037378785227,21.3070607263234,-18.0445099944961));
#46249=CARTESIAN_POINT('Ctrl Pts',(20.2341639522258,21.2857262523482,-18.0463627697139));
#46250=CARTESIAN_POINT('Ctrl Pts',(20.2641061444964,21.2637426544939,-18.0482155449317));
#46251=CARTESIAN_POINT('Ctrl Pts',(20.2935358855687,21.2411349269503,-18.0500683201495));
#46252=CARTESIAN_POINT('Ctrl Pts',(20.2917780654112,21.2388105542776,-17.2500265414872));
#46253=CARTESIAN_POINT('Ctrl Pts',(20.5375805895458,21.0526898515823,-17.2653209305498));
#46254=CARTESIAN_POINT('Ctrl Pts',(21.3400060558233,20.1920438331041,-17.3230072551729));
#46255=CARTESIAN_POINT('Ctrl Pts',(21.4691813416985,17.9140516551704,-17.4230855153565));
#46256=CARTESIAN_POINT('Ctrl Pts',(19.1239734719678,16.2091318029775,-17.550261322038));
#46257=CARTESIAN_POINT('Ctrl Pts',(16.6895185666654,17.1540155201862,-17.6648027803286));
#46258=CARTESIAN_POINT('Ctrl Pts',(16.1805385807744,18.6141143559075,-17.7369523030588));
#46259=CARTESIAN_POINT('Ctrl Pts',(16.1756125809373,19.2132129985223,-17.7667098902285));
#46260=CARTESIAN_POINT('Origin',(18.734,19.211,1.76670989022852));
#46261=CARTESIAN_POINT('',(20.2935358855687,21.2411349269503,-16.4501666916289));
#46262=CARTESIAN_POINT('',(20.2935358855687,21.2411349269503,-16.5166303570915));
#46263=CARTESIAN_POINT('',(20.2935358855687,21.2411349269503,1.76670989022852));
#46264=CARTESIAN_POINT('',(16.1737370555978,19.211835565301,-17.0332901097715));
#46265=CARTESIAN_POINT('Ctrl Pts',(20.2935358855687,21.2411349269503,-16.5166303570915));
#46266=CARTESIAN_POINT('Ctrl Pts',(20.36010259041,21.1899988356463,-16.5208151874521));
#46267=CARTESIAN_POINT('Ctrl Pts',(20.4240566305495,21.1356583062745,-16.5250000178127));
#46268=CARTESIAN_POINT('Ctrl Pts',(20.4850922765871,21.078424921885,-16.5291848481734));
#46269=CARTESIAN_POINT('Ctrl Pts',(20.4960575744632,21.0681427155182,-16.5299366696817));
#46270=CARTESIAN_POINT('Ctrl Pts',(20.5069287828259,21.0577672286989,-16.53068849119));
#46271=CARTESIAN_POINT('Ctrl Pts',(20.5177042670233,21.0473003806031,-16.5314403126983));
#46272=CARTESIAN_POINT('Ctrl Pts',(20.5776805529837,20.9890419614915,-16.5356249470914));
#46273=CARTESIAN_POINT('Ctrl Pts',(20.6349112416909,20.9277336646777,-16.5398095814844));
#46274=CARTESIAN_POINT('Ctrl Pts',(20.6890701824651,20.8636646912292,-16.5439942158775));
#46275=CARTESIAN_POINT('Ctrl Pts',(20.7431520346907,20.7996869120343,-16.5481728939614));
#46276=CARTESIAN_POINT('Ctrl Pts',(20.7941705292094,20.7329566097132,-16.5523515720454));
#46277=CARTESIAN_POINT('Ctrl Pts',(20.8418355824982,20.6638004533157,-16.5565302501293));
#46278=CARTESIAN_POINT('Ctrl Pts',(20.890354997611,20.5934047225164,-16.5607838280147));
#46279=CARTESIAN_POINT('Ctrl Pts',(20.9353992222982,20.5204956513051,-16.5650374059002));
#46280=CARTESIAN_POINT('Ctrl Pts',(20.9767045339426,20.4454538765922,-16.5692909837856));
#46281=CARTESIAN_POINT('Ctrl Pts',(21.01720906152,20.371866933114,-16.5734620977636));
#46282=CARTESIAN_POINT('Ctrl Pts',(21.0541181225501,20.2962296630072,-16.5776332117415));
#46283=CARTESIAN_POINT('Ctrl Pts',(21.0872271712958,20.2189295016395,-16.5818043257195));
#46284=CARTESIAN_POINT('Ctrl Pts',(21.1203251099804,20.1416552790874,-16.5859740400399));
#46285=CARTESIAN_POINT('Ctrl Pts',(21.149625387836,20.0627196959936,-16.5901437543602));
#46286=CARTESIAN_POINT('Ctrl Pts',(21.1749707834402,19.9825320047745,-16.5943134686806));
#46287=CARTESIAN_POINT('Ctrl Pts',(21.2003152771464,19.9023471669775,-16.5984830346247));
#46288=CARTESIAN_POINT('Ctrl Pts',(21.2217050305799,19.8209107485431,-16.6026526005687));
#46289=CARTESIAN_POINT('Ctrl Pts',(21.2390325027795,19.7386477613126,-16.6068221665128));
#46290=CARTESIAN_POINT('Ctrl Pts',(21.2569691875259,19.6534925089337,-16.6111383292517));
#46291=CARTESIAN_POINT('Ctrl Pts',(21.2705525077455,19.5674519980823,-16.6154544919906));
#46292=CARTESIAN_POINT('Ctrl Pts',(21.2797210678871,19.4810078600997,-16.6197706547295));
#46293=CARTESIAN_POINT('Ctrl Pts',(21.2885909631466,19.3973796308195,-16.6239462189212));
#46294=CARTESIAN_POINT('Ctrl Pts',(21.2933293236125,19.3133741398417,-16.6281217831129));
#46295=CARTESIAN_POINT('Ctrl Pts',(21.2939336612287,19.2294295987025,-16.6322973473046));
#46296=CARTESIAN_POINT('Ctrl Pts',(21.2945685225012,19.1412452183497,-16.6366838093171));
#46297=CARTESIAN_POINT('Ctrl Pts',(21.2906407927078,19.0531286901045,-16.6410702713296));
#46298=CARTESIAN_POINT('Ctrl Pts',(21.2822091879386,18.965582122686,-16.6454567333422));
#46299=CARTESIAN_POINT('Ctrl Pts',(21.2737775831694,18.8780355552674,-16.6498431953547));
#46300=CARTESIAN_POINT('Ctrl Pts',(21.2608422640145,18.7910595113906,-16.6542296573673));
#46301=CARTESIAN_POINT('Ctrl Pts',(21.2435233083642,18.7051415565825,-16.6586161193798));
#46302=CARTESIAN_POINT('Ctrl Pts',(21.2270012235363,18.6231768142361,-16.6628007537728));
#46303=CARTESIAN_POINT('Ctrl Pts',(21.2064285344955,18.5418698437248,-16.6669853881659));
#46304=CARTESIAN_POINT('Ctrl Pts',(21.1818718743958,18.4616514252084,-16.6711700225589));
#46305=CARTESIAN_POINT('Ctrl Pts',(21.1573501676622,18.3815471876817,-16.6753487006429));
#46306=CARTESIAN_POINT('Ctrl Pts',(21.1288558871502,18.3025288606373,-16.6795273787268));
#46307=CARTESIAN_POINT('Ctrl Pts',(21.0965066931249,18.2250171781719,-16.6837060568108));
#46308=CARTESIAN_POINT('Ctrl Pts',(21.0635776630457,18.146116154505,-16.6879596346962));
#46309=CARTESIAN_POINT('Ctrl Pts',(21.0266542567595,18.0687767925293,-16.6922132125816));
#46310=CARTESIAN_POINT('Ctrl Pts',(20.9859137816201,17.9934268727713,-16.6964667904671));
#46311=CARTESIAN_POINT('Ctrl Pts',(20.9459631400899,17.9195377582412,-16.700637904445));
#46312=CARTESIAN_POINT('Ctrl Pts',(20.9023423404875,17.847562059166,-16.704809018423));
#46313=CARTESIAN_POINT('Ctrl Pts',(20.8552664379162,17.7778814775567,-16.7089801324009));
#46314=CARTESIAN_POINT('Ctrl Pts',(20.8082063321188,17.7082242779395,-16.7131498467213));
#46315=CARTESIAN_POINT('Ctrl Pts',(20.7576936832433,17.6408610471354,-16.7173195610417));
#46316=CARTESIAN_POINT('Ctrl Pts',(20.7039875068324,17.5761455040511,-16.721489275362));
#46317=CARTESIAN_POINT('Ctrl Pts',(20.6502832415178,17.5114322638236,-16.7256588413061));
#46318=CARTESIAN_POINT('Ctrl Pts',(20.5933859690518,17.4493668774532,-16.7298284072501));
#46319=CARTESIAN_POINT('Ctrl Pts',(20.5335948472512,17.3902698207184,-16.7339979731942));
#46320=CARTESIAN_POINT('Ctrl Pts',(20.4717015433684,17.3290949843729,-16.7383141359331));
#46321=CARTESIAN_POINT('Ctrl Pts',(20.4067074835552,17.2711014650386,-16.742630298672));
#46322=CARTESIAN_POINT('Ctrl Pts',(20.3389844113023,17.2166015845683,-16.7469464614109));
#46323=CARTESIAN_POINT('Ctrl Pts',(20.273467411005,17.1638770319719,-16.7511220256026));
#46324=CARTESIAN_POINT('Ctrl Pts',(20.2053968718999,17.1144222417057,-16.7552975897943));
#46325=CARTESIAN_POINT('Ctrl Pts',(20.135139913803,17.0684765014245,-16.759473153986));
#46326=CARTESIAN_POINT('Ctrl Pts',(20.0613344437726,17.0202101510273,-16.7638596159985));
#46327=CARTESIAN_POINT('Ctrl Pts',(19.9851163826193,16.9758169447297,-16.7682460780111));
#46328=CARTESIAN_POINT('Ctrl Pts',(19.9069397062212,16.9355192935185,-16.7726325400236));
#46329=CARTESIAN_POINT('Ctrl Pts',(19.8287630298231,16.8952216423072,-16.7770190020362));
#46330=CARTESIAN_POINT('Ctrl Pts',(19.7486282982591,16.8590197157384,-16.7814054640487));
#46331=CARTESIAN_POINT('Ctrl Pts',(19.6670104728629,16.8270764572814,-16.7857919260613));
#46332=CARTESIAN_POINT('Ctrl Pts',(19.5891480046,16.7966029554973,-16.7899765604543));
#46333=CARTESIAN_POINT('Ctrl Pts',(19.5096461031212,16.7698914102528,-16.7941611948473));
#46334=CARTESIAN_POINT('Ctrl Pts',(19.4289030536308,16.7471189667408,-16.7983458292404));
#46335=CARTESIAN_POINT('Ctrl Pts',(19.3482749318773,16.7243789369834,-16.8025245073243));
#46336=CARTESIAN_POINT('Ctrl Pts',(19.2664096101499,16.7055669958483,-16.8067031854083));
#46337=CARTESIAN_POINT('Ctrl Pts',(19.1837245465113,16.6908119450594,-16.8108818634922));
#46338=CARTESIAN_POINT('Ctrl Pts',(19.0995574125317,16.6757924205894,-16.8151354413777));
#46339=CARTESIAN_POINT('Ctrl Pts',(19.0145413088147,16.66497683224,-16.8193890192631));
#46340=CARTESIAN_POINT('Ctrl Pts',(18.929131904193,16.6584476420716,-16.8236425971485));
#46341=CARTESIAN_POINT('Ctrl Pts',(18.8453783275426,16.6520450329952,-16.8278137111265));
#46342=CARTESIAN_POINT('Ctrl Pts',(18.7612470435307,16.6497641415373,-16.8319848251044));
#46343=CARTESIAN_POINT('Ctrl Pts',(18.6771754083917,16.6516307484483,-16.8361559390824));
#46344=CARTESIAN_POINT('Ctrl Pts',(18.5931319843018,16.6534967290012,-16.8403256534028));
#46345=CARTESIAN_POINT('Ctrl Pts',(18.5091486288698,16.659507433716,-16.8444953677231));
#46346=CARTESIAN_POINT('Ctrl Pts',(18.4256629639197,16.6696365328467,-16.8486650820435));
#46347=CARTESIAN_POINT('Ctrl Pts',(18.3421802697478,16.6797652715406,-16.8528346479875));
#46348=CARTESIAN_POINT('Ctrl Pts',(18.259195687427,16.6940120570168,-16.8570042139316));
#46349=CARTESIAN_POINT('Ctrl Pts',(18.1771406148227,16.7122988123547,-16.8611737798756));
#46350=CARTESIAN_POINT('Ctrl Pts',(18.0922005870916,16.7312285074512,-16.8654899426145));
#46351=CARTESIAN_POINT('Ctrl Pts',(18.008257163138,16.7544874341396,-16.8698061053534));
#46352=CARTESIAN_POINT('Ctrl Pts',(17.9257741739149,16.781932068869,-16.8741222680924));
#46353=CARTESIAN_POINT('Ctrl Pts',(17.8459780593899,16.8084826975088,-16.878297832284));
#46354=CARTESIAN_POINT('Ctrl Pts',(17.7675491154086,16.838950308513,-16.8824733964757));
#46355=CARTESIAN_POINT('Ctrl Pts',(17.690887260014,16.8731557340835,-16.8866489606674));
#46356=CARTESIAN_POINT('Ctrl Pts',(17.6103533965496,16.9090887943838,-16.8910354226799));
#46357=CARTESIAN_POINT('Ctrl Pts',(17.5317703445184,16.9491469214588,-16.8954218846925));
#46358=CARTESIAN_POINT('Ctrl Pts',(17.4555708448952,16.9930687802869,-16.899808346705));
#46359=CARTESIAN_POINT('Ctrl Pts',(17.3793713452719,17.0369906391151,-16.9041948087175));
#46360=CARTESIAN_POINT('Ctrl Pts',(17.3055558437866,17.0847758505362,-16.9085812707301));
#46361=CARTESIAN_POINT('Ctrl Pts',(17.2345184376722,17.1361132454423,-16.9129677327426));
#46362=CARTESIAN_POINT('Ctrl Pts',(17.167299168743,17.1846913445463,-16.9171184300414));
#46363=CARTESIAN_POINT('Ctrl Pts',(17.1023079512147,17.2366370916662,-16.9212691273401));
#46364=CARTESIAN_POINT('Ctrl Pts',(17.0399060592653,17.2917173944502,-16.9254198246388));
#46365=CARTESIAN_POINT('Ctrl Pts',(16.9775932241692,17.3467190893861,-16.9295645982704));
#46366=CARTESIAN_POINT('Ctrl Pts',(16.9178627255451,17.4048461509352,-16.9337093719019));
#46367=CARTESIAN_POINT('Ctrl Pts',(16.8610458812396,17.4658229691466,-16.9378541455334));
#46368=CARTESIAN_POINT('Ctrl Pts',(16.8042942087153,17.5267298438772,-16.9419941649009));
#46369=CARTESIAN_POINT('Ctrl Pts',(16.7504498675423,17.5904796396564,-16.9461341842684));
#46370=CARTESIAN_POINT('Ctrl Pts',(16.6998090154256,17.6567583719781,-16.9502742036359));
#46371=CARTESIAN_POINT('Ctrl Pts',(16.6491995836851,17.7229959813207,-16.9544116543072));
#46372=CARTESIAN_POINT('Ctrl Pts',(16.6017899801563,17.7917590422704,-16.9585491049784));
#46373=CARTESIAN_POINT('Ctrl Pts',(16.5578367768805,17.8626997269368,-16.9626865556497));
#46374=CARTESIAN_POINT('Ctrl Pts',(16.5138971231854,17.9336185425139,-16.9668227308571));
#46375=CARTESIAN_POINT('Ctrl Pts',(16.473412000563,18.0067132510728,-16.9709589060645));
#46376=CARTESIAN_POINT('Ctrl Pts',(16.436594403761,18.0816074524907,-16.9750950812719));
#46377=CARTESIAN_POINT('Ctrl Pts',(16.3997766632185,18.1565019463048,-16.9792312726275));
#46378=CARTESIAN_POINT('Ctrl Pts',(16.3666266817619,18.2331955257885,-16.983367463983));
#46379=CARTESIAN_POINT('Ctrl Pts',(16.3373106052885,18.3112889656799,-16.9875036553386));
#46380=CARTESIAN_POINT('Ctrl Pts',(16.3079666664254,18.3894566266172,-16.9916437777855));
#46381=CARTESIAN_POINT('Ctrl Pts',(16.2824640727846,18.4690263650884,-16.9957839002324));
#46382=CARTESIAN_POINT('Ctrl Pts',(16.2609198329123,18.5495814584111,-16.9999240226793));
#46383=CARTESIAN_POINT('Ctrl Pts',(16.2393648184701,18.6301768384414,-17.0040662156583));
#46384=CARTESIAN_POINT('Ctrl Pts',(16.2217721969232,18.711758096276,-17.0082084086373));
#46385=CARTESIAN_POINT('Ctrl Pts',(16.2082078057625,18.7938983438913,-17.0123506016163));
#46386=CARTESIAN_POINT('Ctrl Pts',(16.194621013815,18.8761742412484,-17.016499635181));
#46387=CARTESIAN_POINT('Ctrl Pts',(16.1850757885661,18.9590105062903,-17.0206486687458));
#46388=CARTESIAN_POINT('Ctrl Pts',(16.1795860271471,19.0419755778186,-17.0247977023105));
#46389=CARTESIAN_POINT('Ctrl Pts',(16.1758404729028,19.0985809841505,-17.0276285047975));
#46390=CARTESIAN_POINT('Ctrl Pts',(16.1739816679355,19.1552463005709,-17.0304593072845));
#46391=CARTESIAN_POINT('Ctrl Pts',(16.1740001363332,19.2118354794422,-17.0332901097715));
#46392=CARTESIAN_POINT('Ctrl Pts',(16.1700998775752,19.2118367523274,-17.0332901097715));
#46393=CARTESIAN_POINT('Ctrl Pts',(16.1699051698649,19.2575742435185,-17.0355745863224));
#46394=CARTESIAN_POINT('Ctrl Pts',(16.1917620114795,20.1518505208751,-17.0802509984337));
#46395=CARTESIAN_POINT('Ctrl Pts',(17.2348044634258,21.8407724883182,-17.1673193461055));
#46396=CARTESIAN_POINT('Ctrl Pts',(19.336908367695,21.880117833012,-17.2595384002944));
#46397=CARTESIAN_POINT('Ctrl Pts',(20.1770115565028,21.3343829456268,-17.3093655189228));
#46398=CARTESIAN_POINT('Ctrl Pts',(20.2944552762683,21.2423103685662,-17.3168007019908));
#46399=CARTESIAN_POINT('',(16.1741505176752,19.209803254934,-16.9667098397549));
#46400=CARTESIAN_POINT('Ctrl Pts',(16.1776746320478,19.209805920766,-16.9667098902285));
#46401=CARTESIAN_POINT('Ctrl Pts',(16.1797896414426,19.7131225343252,-16.9916592919231));
#46402=CARTESIAN_POINT('Ctrl Pts',(16.5671403882425,21.07463612297,-17.0590006291781));
#46403=CARTESIAN_POINT('Ctrl Pts',(18.4733994225959,22.0756037013586,-17.153439512931));
#46404=CARTESIAN_POINT('Ctrl Pts',(19.8562820609774,21.5685664127725,-17.2229289949893));
#46405=CARTESIAN_POINT('Ctrl Pts',(20.2917780654112,21.2388105542776,-17.2500265414872));
#46406=CARTESIAN_POINT('Ctrl Pts',(20.2935358855687,21.2411349269503,-16.4501666916289));
#46407=CARTESIAN_POINT('Ctrl Pts',(20.3601794036991,21.1899398281984,-16.4543369074164));
#46408=CARTESIAN_POINT('Ctrl Pts',(20.424336074523,21.1354315300474,-16.4585071232039));
#46409=CARTESIAN_POINT('Ctrl Pts',(20.4856659995229,21.0778867737802,-16.4626773389914));
#46410=CARTESIAN_POINT('Ctrl Pts',(20.5469851014509,21.0203521726051,-16.4668468188487));
#46411=CARTESIAN_POINT('Ctrl Pts',(20.6054781133613,20.9597824927492,-16.471016298706));
#46412=CARTESIAN_POINT('Ctrl Pts',(20.6608402875572,20.8964929564512,-16.4751857785632));
#46413=CARTESIAN_POINT('Ctrl Pts',(20.7162092989616,20.8331956039182,-16.4793557733498));
#46414=CARTESIAN_POINT('Ctrl Pts',(20.7684464030089,20.7671780750758,-16.4835257681363));
#46415=CARTESIAN_POINT('Ctrl Pts',(20.8172865168588,20.6987893966131,-16.4876957629229));
#46416=CARTESIAN_POINT('Ctrl Pts',(20.8661791232192,20.6303272151803,-16.4918702395478));
#46417=CARTESIAN_POINT('Ctrl Pts',(20.911667183017,20.5594891716793,-16.4960447161727));
#46418=CARTESIAN_POINT('Ctrl Pts',(20.9535287381871,20.4866536286788,-16.5002191927976));
#46419=CARTESIAN_POINT('Ctrl Pts',(20.9954147198633,20.413775585637,-16.5043961052584));
#46420=CARTESIAN_POINT('Ctrl Pts',(21.0336697749439,20.3388981323474,-16.5085730177192));
#46421=CARTESIAN_POINT('Ctrl Pts',(21.068118859428,20.2624224412968,-16.5127499301799));
#46422=CARTESIAN_POINT('Ctrl Pts',(21.1026261826924,20.185817462312,-16.5169339040268));
#46423=CARTESIAN_POINT('Ctrl Pts',(21.1333145201899,20.107609278805,-16.5211178778737));
#46424=CARTESIAN_POINT('Ctrl Pts',(21.1600578409485,20.0282168331431,-16.5253018517207));
#46425=CARTESIAN_POINT('Ctrl Pts',(21.1761504170598,19.9804430736308,-16.5278195240093));
#46426=CARTESIAN_POINT('Ctrl Pts',(21.1908155024365,19.9322407738411,-16.5303371962979));
#46427=CARTESIAN_POINT('Ctrl Pts',(21.2040345704695,19.8837029215676,-16.5328548685865));
#46428=CARTESIAN_POINT('Ctrl Pts',(21.2260060426842,19.8030279397969,-16.5370395029795));
#46429=CARTESIAN_POINT('Ctrl Pts',(21.244061800264,19.7211252621464,-16.5412241373726));
#46430=CARTESIAN_POINT('Ctrl Pts',(21.2580683099057,19.6384098348539,-16.5454087717656));
#46431=CARTESIAN_POINT('Ctrl Pts',(21.2720548830146,19.555812142734,-16.5495874498496));
#46432=CARTESIAN_POINT('Ctrl Pts',(21.2820035803663,19.4724044485338,-16.5537661279335));
#46433=CARTESIAN_POINT('Ctrl Pts',(21.28783098536,19.3886155911377,-16.5579448060175));
#46434=CARTESIAN_POINT('Ctrl Pts',(21.2937628424001,19.3033248786908,-16.5621983839029));
#46435=CARTESIAN_POINT('Ctrl Pts',(21.2954240788116,19.2176396691377,-16.5664519617883));
#46436=CARTESIAN_POINT('Ctrl Pts',(21.2927814384536,19.1320218370346,-16.5707055396738));
#46437=CARTESIAN_POINT('Ctrl Pts',(21.2901900308356,19.0480638736762,-16.5748766536517));
#46438=CARTESIAN_POINT('Ctrl Pts',(21.2834601502021,18.9641711795843,-16.5790477676297));
#46439=CARTESIAN_POINT('Ctrl Pts',(21.2726129381323,18.8807813597822,-16.5832188816076));
#46440=CARTESIAN_POINT('Ctrl Pts',(21.2617693659493,18.7974195222394,-16.587388595928));
#46441=CARTESIAN_POINT('Ctrl Pts',(21.246811265521,18.7145606796674,-16.5915583102484));
#46442=CARTESIAN_POINT('Ctrl Pts',(21.2278116184524,18.6326371280314,-16.5957280245688));
#46443=CARTESIAN_POINT('Ctrl Pts',(21.2088126474729,18.550716491587,-16.5998975905128));
#46444=CARTESIAN_POINT('Ctrl Pts',(21.1857725205575,18.4697315278524,-16.6040671564568));
#46445=CARTESIAN_POINT('Ctrl Pts',(21.1588150040535,18.3901028102636,-16.6082367224009));
#46446=CARTESIAN_POINT('Ctrl Pts',(21.1309096945249,18.3076744451972,-16.6125528851398));
#46447=CARTESIAN_POINT('Ctrl Pts',(21.0988065683011,18.2266999715501,-16.6168690478787));
#46448=CARTESIAN_POINT('Ctrl Pts',(21.0626979316573,18.1476252104291,-16.6211852106176));
#46449=CARTESIAN_POINT('Ctrl Pts',(21.0277655300542,18.0711263013344,-16.6253607748093));
#46450=CARTESIAN_POINT('Ctrl Pts',(20.9890848280186,17.9964056357567,-16.629536339001));
#46451=CARTESIAN_POINT('Ctrl Pts',(20.9468767362673,17.9238416763711,-16.6337119031927));
#46452=CARTESIAN_POINT('Ctrl Pts',(20.9025368141418,17.8476126839013,-16.6380983652052));
#46453=CARTESIAN_POINT('Ctrl Pts',(20.854304119971,17.7737644826752,-16.6424848272178));
#46454=CARTESIAN_POINT('Ctrl Pts',(20.8024847707862,17.702699382409,-16.6468712892303));
#46455=CARTESIAN_POINT('Ctrl Pts',(20.7506654216015,17.6316342821428,-16.6512577512428));
#46456=CARTESIAN_POINT('Ctrl Pts',(20.6952598420585,17.5633526854596,-16.6556442132554));
#46457=CARTESIAN_POINT('Ctrl Pts',(20.6366195645773,17.4982131503051,-16.6600306752679));
#46458=CARTESIAN_POINT('Ctrl Pts',(20.5806774131887,17.4360707817229,-16.664215309661));
#46459=CARTESIAN_POINT('Ctrl Pts',(20.5215834617877,17.3765563809788,-16.668399944054));
#46460=CARTESIAN_POINT('Ctrl Pts',(20.4596143354494,17.3200068309771,-16.6725845784471));
#46461=CARTESIAN_POINT('Ctrl Pts',(20.3977334144923,17.2635377722604,-16.676763256531));
#46462=CARTESIAN_POINT('Ctrl Pts',(20.3329857844083,17.2100254892845,-16.6809419346149));
#46463=CARTESIAN_POINT('Ctrl Pts',(20.26568687901,17.1597722445646,-16.6851206126989));
#46464=CARTESIAN_POINT('Ctrl Pts',(20.1971816890993,17.1086182465494,-16.6893741905843));
#46465=CARTESIAN_POINT('Ctrl Pts',(20.1260331836052,17.0608416308411,-16.6936277684697));
#46466=CARTESIAN_POINT('Ctrl Pts',(20.052611725018,17.0167203645284,-16.6978813463552));
#46467=CARTESIAN_POINT('Ctrl Pts',(19.9806136846756,16.9734544750588,-16.7020524603331));
#46468=CARTESIAN_POINT('Ctrl Pts',(19.9064304485064,16.9337037154837,-16.7062235743111));
#46469=CARTESIAN_POINT('Ctrl Pts',(19.8304414166181,16.89768717638,-16.710394688289));
#46470=CARTESIAN_POINT('Ctrl Pts',(19.7544778835833,16.8616827229739,-16.7145644026094));
#46471=CARTESIAN_POINT('Ctrl Pts',(19.6767101736173,16.8294101983214,-16.7187341169298));
#46472=CARTESIAN_POINT('Ctrl Pts',(19.5975412827732,16.8010422300492,-16.7229038312502));
#46473=CARTESIAN_POINT('Ctrl Pts',(19.518375209098,16.772675271231,-16.7270733971942));
#46474=CARTESIAN_POINT('Ctrl Pts',(19.4378084870369,16.7482127469195,-16.7312429631383));
#46475=CARTESIAN_POINT('Ctrl Pts',(19.3562617446687,16.7277782376272,-16.7354125290823));
#46476=CARTESIAN_POINT('Ctrl Pts',(19.2718479194376,16.7066252761968,-16.7397286918212));
#46477=CARTESIAN_POINT('Ctrl Pts',(19.1863843882477,16.6897889781384,-16.7440448545601));
#46478=CARTESIAN_POINT('Ctrl Pts',(19.1003501078363,16.6773489588169,-16.748361017299));
#46479=CARTESIAN_POINT('Ctrl Pts',(19.0171183850602,16.6653141718163,-16.7525365814907));
#46480=CARTESIAN_POINT('Ctrl Pts',(18.9333529997369,16.6573936417868,-16.7567121456824));
#46481=CARTESIAN_POINT('Ctrl Pts',(18.849491753864,16.6536064724432,-16.7608877098741));
#46482=CARTESIAN_POINT('Ctrl Pts',(18.761394875823,16.6496280221792,-16.7652741718866));
#46483=CARTESIAN_POINT('Ctrl Pts',(18.6731927827737,16.6502114543057,-16.7696606338992));
#46484=CARTESIAN_POINT('Ctrl Pts',(18.5853894488637,16.6553171354624,-16.7740470959117));
#46485=CARTESIAN_POINT('Ctrl Pts',(18.4975861149538,16.6604228166191,-16.7784335579242));
#46486=CARTESIAN_POINT('Ctrl Pts',(18.4101821085833,16.6700506076701,-16.7828200199368));
#46487=CARTESIAN_POINT('Ctrl Pts',(18.3236691980735,16.6840990060965,-16.7872064819493));
#46488=CARTESIAN_POINT('Ctrl Pts',(18.2411368748191,16.6975010168866,-16.7913911163424));
#46489=CARTESIAN_POINT('Ctrl Pts',(18.1591082470637,16.7149756618514,-16.7955757507354));
#46490=CARTESIAN_POINT('Ctrl Pts',(18.0780163119231,16.7364726914061,-16.7997603851285));
#46491=CARTESIAN_POINT('Ctrl Pts',(17.9970398011148,16.7579391226001,-16.8039390632124));
#46492=CARTESIAN_POINT('Ctrl Pts',(17.9169977755057,16.7834164491322,-16.8081177412964));
#46493=CARTESIAN_POINT('Ctrl Pts',(17.838315128377,16.8128030500508,-16.8122964193803));
#46494=CARTESIAN_POINT('Ctrl Pts',(17.7582221513469,16.8427163846711,-16.8165499972658));
#46495=CARTESIAN_POINT('Ctrl Pts',(17.6795382417638,16.8766804423688,-16.8208035751512));
#46496=CARTESIAN_POINT('Ctrl Pts',(17.6026975961515,16.9145342652139,-16.8250571530366));
#46497=CARTESIAN_POINT('Ctrl Pts',(17.5273466563965,16.9516542178375,-16.8292282670146));
#46498=CARTESIAN_POINT('Ctrl Pts',(17.453768579546,16.992514247479,-16.8333993809925));
#46499=CARTESIAN_POINT('Ctrl Pts',(17.3823529481855,17.0369139282629,-16.8375704949705));
#46500=CARTESIAN_POINT('Ctrl Pts',(17.31096128103,17.0812987103051,-16.8417402092909));
#46501=CARTESIAN_POINT('Ctrl Pts',(17.2417310086118,17.1292205418819,-16.8459099236112));
#46502=CARTESIAN_POINT('Ctrl Pts',(17.1750254175661,17.1804340071485,-16.8500796379316));
#46503=CARTESIAN_POINT('Ctrl Pts',(17.1083222001915,17.2316456500203,-16.8542492038757));
#46504=CARTESIAN_POINT('Ctrl Pts',(17.0441438499408,17.2861484128723,-16.8584187698197));
#46505=CARTESIAN_POINT('Ctrl Pts',(16.9828219564695,17.3436555058435,-16.8625883357637));
#46506=CARTESIAN_POINT('Ctrl Pts',(16.9193440608725,17.4031844772608,-16.8669044985027));
#46507=CARTESIAN_POINT('Ctrl Pts',(16.8589276101183,17.4659326132811,-16.8712206612416));
#46508=CARTESIAN_POINT('Ctrl Pts',(16.8018987983271,17.5315402813719,-16.8755368239805));
#46509=CARTESIAN_POINT('Ctrl Pts',(16.7467276940816,17.5950107865755,-16.8797123881722));
#46510=CARTESIAN_POINT('Ctrl Pts',(16.6947271674384,17.6611569867928,-16.8838879523639));
#46511=CARTESIAN_POINT('Ctrl Pts',(16.6461502555162,17.729621100306,-16.8880635165556));
#46512=CARTESIAN_POINT('Ctrl Pts',(16.5951198392535,17.8015431734345,-16.8924499785681));
#46513=CARTESIAN_POINT('Ctrl Pts',(16.5478682932593,17.8760229761494,-16.8968364405807));
#46514=CARTESIAN_POINT('Ctrl Pts',(16.5046350837971,17.952615293162,-16.9012229025932));
#46515=CARTESIAN_POINT('Ctrl Pts',(16.4614018743349,18.0292076101746,-16.9056093646057));
#46516=CARTESIAN_POINT('Ctrl Pts',(16.4221871920777,18.1079118882385,-16.9099958266183));
#46517=CARTESIAN_POINT('Ctrl Pts',(16.3871718743353,18.1882596866316,-16.9143822886308));
#46518=CARTESIAN_POINT('Ctrl Pts',(16.3503471043862,18.272759539339,-16.9189954255354));
#46519=CARTESIAN_POINT('Ctrl Pts',(16.3180481684135,18.3593459986726,-16.9236085624399));
#46520=CARTESIAN_POINT('Ctrl Pts',(16.2904920397068,18.4475415217682,-16.9282216993445));
#46521=CARTESIAN_POINT('Ctrl Pts',(16.2630147812854,18.5354846144106,-16.9328216326736));
#46522=CARTESIAN_POINT('Ctrl Pts',(16.240253377301,18.6250273148911,-16.9374215660027));
#46523=CARTESIAN_POINT('Ctrl Pts',(16.2223767943066,18.7156729639699,-16.9420214993319));
#46524=CARTESIAN_POINT('Ctrl Pts',(16.2045882581335,18.8058721596483,-16.9465987767929));
#46525=CARTESIAN_POINT('Ctrl Pts',(16.1916366671697,18.8971631896627,-16.9511760542538));
#46526=CARTESIAN_POINT('Ctrl Pts',(16.1836406660146,18.9890376888893,-16.9557533317148));
#46527=CARTESIAN_POINT('Ctrl Pts',(16.1772607284144,19.0623435277384,-16.9594055003442));
#46528=CARTESIAN_POINT('Ctrl Pts',(16.174034774907,19.1360203999197,-16.9630576689737));
#46529=CARTESIAN_POINT('Ctrl Pts',(16.1740002797795,19.2098031412859,-16.9667098376031));
#46530=CARTESIAN_POINT('Origin',(18.734,19.211,1.76670989022852));
#46531=CARTESIAN_POINT('',(20.2958871626529,21.2441650537926,-15.6501589834813));
#46532=CARTESIAN_POINT('',(20.2935358855687,21.2411349269503,-15.7166572087383));
#46533=CARTESIAN_POINT('',(20.2935358855687,21.2411349269503,1.76670989022852));
#46534=CARTESIAN_POINT('',(16.1740007055014,19.2129005700936,-16.2332901098004));
#46535=CARTESIAN_POINT('Ctrl Pts',(20.2935358855687,21.2411349269503,-15.7166572087383));
#46536=CARTESIAN_POINT('Ctrl Pts',(20.3624598532065,21.1881880023494,-15.7209678973943));
#46537=CARTESIAN_POINT('Ctrl Pts',(20.4286597734137,21.131746121533,-15.7252785860502));
#46538=CARTESIAN_POINT('Ctrl Pts',(20.4917771246324,21.0721339500743,-15.7295892747062));
#46539=CARTESIAN_POINT('Ctrl Pts',(20.5529161163786,21.0143902712218,-15.7337648485075));
#46540=CARTESIAN_POINT('Ctrl Pts',(20.6111626397197,20.9536724844389,-15.7379404223088));
#46541=CARTESIAN_POINT('Ctrl Pts',(20.6662297645119,20.8903118046195,-15.7421159961101));
#46542=CARTESIAN_POINT('Ctrl Pts',(20.7239697147345,20.8238757502104,-15.7464942421934));
#46543=CARTESIAN_POINT('Ctrl Pts',(20.7782134501061,20.7545341994174,-15.7508724882766));
#46544=CARTESIAN_POINT('Ctrl Pts',(20.8286804984858,20.6827043212763,-15.7552507343599));
#46545=CARTESIAN_POINT('Ctrl Pts',(20.8791475468655,20.6108744431352,-15.7596289804432));
#46546=CARTESIAN_POINT('Ctrl Pts',(20.9258376663792,20.5365567644941,-15.7640072265265));
#46547=CARTESIAN_POINT('Ctrl Pts',(20.968526025902,20.4601971179788,-15.7683854726097));
#46548=CARTESIAN_POINT('Ctrl Pts',(21.0093266510939,20.3872141935449,-15.7725701070028));
#46549=CARTESIAN_POINT('Ctrl Pts',(21.0466238491571,20.3120944357929,-15.7767547413958));
#46550=CARTESIAN_POINT('Ctrl Pts',(21.0801878476018,20.235208271674,-15.7809393757889));
#46551=CARTESIAN_POINT('Ctrl Pts',(21.1137040718491,20.1584315454932,-15.7851180538728));
#46552=CARTESIAN_POINT('Ctrl Pts',(21.1434974687763,20.0798938250633,-15.7892967319567));
#46553=CARTESIAN_POINT('Ctrl Pts',(21.1693835453414,19.9999911197727,-15.7934754100407));
#46554=CARTESIAN_POINT('Ctrl Pts',(21.195733611225,19.9186562159148,-15.7977289879261));
#46555=CARTESIAN_POINT('Ctrl Pts',(21.218034666248,19.8359073320104,-15.8019825658116));
#46556=CARTESIAN_POINT('Ctrl Pts',(21.2361429171342,19.7521846470801,-15.806236143697));
#46557=CARTESIAN_POINT('Ctrl Pts',(21.2539001042416,19.6700850897685,-15.8104072576749));
#46558=CARTESIAN_POINT('Ctrl Pts',(21.2676255061034,19.5870496228941,-15.8145783716529));
#46559=CARTESIAN_POINT('Ctrl Pts',(21.2772339776254,19.5035080085254,-15.8187494856308));
#46560=CARTESIAN_POINT('Ctrl Pts',(21.2868392249321,19.4199944273523,-15.8229191999512));
#46561=CARTESIAN_POINT('Ctrl Pts',(21.2923302330118,19.3359754926349,-15.8270889142716));
#46562=CARTESIAN_POINT('Ctrl Pts',(21.2936734448665,19.2518883314074,-15.8312586285919));
#46563=CARTESIAN_POINT('Ctrl Pts',(21.295016608924,19.1678041623622,-15.835428194536));
#46564=CARTESIAN_POINT('Ctrl Pts',(21.2922122637205,19.0836522316218,-15.83959776048));
#46565=CARTESIAN_POINT('Ctrl Pts',(21.2852789648471,18.9998705526723,-15.8437673264241));
#46566=CARTESIAN_POINT('Ctrl Pts',(21.2781018997384,18.9131432132467,-15.848083489163));
#46567=CARTESIAN_POINT('Ctrl Pts',(21.2665001742354,18.8268131717716,-15.8523996519019));
#46568=CARTESIAN_POINT('Ctrl Pts',(21.2505527597976,18.7413594915736,-15.8567158146408));
#46569=CARTESIAN_POINT('Ctrl Pts',(21.2351248307078,18.6586894560199,-15.8608913788325));
#46570=CARTESIAN_POINT('Ctrl Pts',(21.2156301415437,18.576840010886,-15.8650669430242));
#46571=CARTESIAN_POINT('Ctrl Pts',(21.1921916857821,18.4962317606722,-15.8692425072158));
#46572=CARTESIAN_POINT('Ctrl Pts',(21.1675694093397,18.4115521793681,-15.8736289692284));
#46573=CARTESIAN_POINT('Ctrl Pts',(21.138594688676,18.3282430251666,-15.8780154312409));
#46574=CARTESIAN_POINT('Ctrl Pts',(21.1054674445919,18.246768617374,-15.8824018932535));
#46575=CARTESIAN_POINT('Ctrl Pts',(21.0723402005078,18.1652942095814,-15.886788355266));
#46576=CARTESIAN_POINT('Ctrl Pts',(21.0350607478797,18.0856550414426,-15.8911748172785));
#46577=CARTESIAN_POINT('Ctrl Pts',(20.9938836431738,18.0082839406927,-15.8955612792911));
#46578=CARTESIAN_POINT('Ctrl Pts',(20.9546011580944,17.9344727989798,-15.8997459136841));
#46579=CARTESIAN_POINT('Ctrl Pts',(20.9116255956987,17.8624508577059,-15.9039305480772));
#46580=CARTESIAN_POINT('Ctrl Pts',(20.8651440549406,17.7926118242556,-15.9081151824702));
#46581=CARTESIAN_POINT('Ctrl Pts',(20.8187286749023,17.722872198025,-15.9122938605542));
#46582=CARTESIAN_POINT('Ctrl Pts',(20.7688174815647,17.6553096876334,-15.9164725386381));
#46583=CARTESIAN_POINT('Ctrl Pts',(20.7156435935689,17.5902937749033,-15.9206512167221));
#46584=CARTESIAN_POINT('Ctrl Pts',(20.6615166018463,17.5241124986637,-15.9249047946075));
#46585=CARTESIAN_POINT('Ctrl Pts',(20.6040090238884,17.4605704392069,-15.9291583724929));
#46586=CARTESIAN_POINT('Ctrl Pts',(20.5434131480187,17.4000267644779,-15.9334119503784));
#46587=CARTESIAN_POINT('Ctrl Pts',(20.4839920414458,17.3406568470248,-15.9375830643563));
#46588=CARTESIAN_POINT('Ctrl Pts',(20.4216016541568,17.2841704328241,-15.9417541783343));
#46589=CARTESIAN_POINT('Ctrl Pts',(20.3565572606157,17.2308717374818,-15.9459252923122));
#46590=CARTESIAN_POINT('Ctrl Pts',(20.291534693349,17.1775909270315,-15.9500950066326));
#46591=CARTESIAN_POINT('Ctrl Pts',(20.2238602440646,17.1274960023899,-15.954264720953));
#46592=CARTESIAN_POINT('Ctrl Pts',(20.153883303655,17.0808517882547,-15.9584344352734));
#46593=CARTESIAN_POINT('Ctrl Pts',(20.0839088533252,17.0342092339207,-15.9626040012174));
#46594=CARTESIAN_POINT('Ctrl Pts',(20.0116324580342,16.9910174003974,-15.9667735671615));
#46595=CARTESIAN_POINT('Ctrl Pts',(19.9374324615958,16.9514977737614,-15.9709431331055));
#46596=CARTESIAN_POINT('Ctrl Pts',(19.8606236848184,16.9105886858056,-15.9752592958444));
#46597=CARTESIAN_POINT('Ctrl Pts',(19.7817539879923,16.8736150868689,-15.9795754585834));
#46598=CARTESIAN_POINT('Ctrl Pts',(19.7012689333153,16.8407698823441,-15.9838916213223));
#46599=CARTESIAN_POINT('Ctrl Pts',(19.623405670829,16.808994606902,-15.988067185514));
#46600=CARTESIAN_POINT('Ctrl Pts',(19.5440311349285,16.7810830031342,-15.9922427497056));
#46601=CARTESIAN_POINT('Ctrl Pts',(19.4635655614727,16.7571593182293,-15.9964183138973));
#46602=CARTESIAN_POINT('Ctrl Pts',(19.3790358631902,16.7320273048729,-16.0008047759099));
#46603=CARTESIAN_POINT('Ctrl Pts',(19.2933025817199,16.711296794516,-16.0051912379224));
#46604=CARTESIAN_POINT('Ctrl Pts',(19.206864349456,16.6950510126369,-16.009577699935));
#46605=CARTESIAN_POINT('Ctrl Pts',(19.120426117192,16.6788052307578,-16.0139641619475));
#46606=CARTESIAN_POINT('Ctrl Pts',(19.0332835193118,16.6670441795795,-16.01835062396));
#46607=CARTESIAN_POINT('Ctrl Pts',(18.9459382820314,16.6597880988421,-16.0227370859726));
#46608=CARTESIAN_POINT('Ctrl Pts',(18.8626119285951,16.6528658811356,-16.0269217203656));
#46609=CARTESIAN_POINT('Ctrl Pts',(18.7787910168743,16.6500174172728,-16.0311063547587));
#46610=CARTESIAN_POINT('Ctrl Pts',(18.6949078655891,16.6512984929826,-16.0352909891517));
#46611=CARTESIAN_POINT('Ctrl Pts',(18.6111441115869,16.6525777452396,-16.0394696672357));
#46612=CARTESIAN_POINT('Ctrl Pts',(18.5273187500335,16.6579748547684,-16.0436483453196));
#46613=CARTESIAN_POINT('Ctrl Pts',(18.4438686393691,16.6674937991862,-16.0478270234036));
#46614=CARTESIAN_POINT('Ctrl Pts',(18.3589227454458,16.6771833638415,-16.052080601289));
#46615=CARTESIAN_POINT('Ctrl Pts',(18.2743661679605,16.6911440245191,-16.0563341791744));
#46616=CARTESIAN_POINT('Ctrl Pts',(18.1906591204412,16.7093244237911,-16.0605877570599));
#46617=CARTESIAN_POINT('Ctrl Pts',(18.1085748973787,16.7271523605471,-16.0647588710378));
#46618=CARTESIAN_POINT('Ctrl Pts',(18.0273080288925,16.749037778107,-16.0689299850158));
#46619=CARTESIAN_POINT('Ctrl Pts',(17.9472849642517,16.7748802466776,-16.0731010989937));
#46620=CARTESIAN_POINT('Ctrl Pts',(17.8672887521232,16.8007140435583,-16.0772708133141));
#46621=CARTESIAN_POINT('Ctrl Pts',(17.7885359523433,16.8305021131095,-16.0814405276345));
#46622=CARTESIAN_POINT('Ctrl Pts',(17.7114383592365,16.8640940174692,-16.0856102419549));
#46623=CARTESIAN_POINT('Ctrl Pts',(17.6343435095929,16.8976847264847,-16.0897798078989));
#46624=CARTESIAN_POINT('Ctrl Pts',(17.5589041709149,16.9350788166486,-16.0939493738429));
#46625=CARTESIAN_POINT('Ctrl Pts',(17.4855113682728,16.9760780469001,-16.098118939787));
#46626=CARTESIAN_POINT('Ctrl Pts',(17.4095381652295,17.0185187595092,-16.1024351025259));
#46627=CARTESIAN_POINT('Ctrl Pts',(17.3357585487129,17.0648225852952,-16.1067512652648));
#46628=CARTESIAN_POINT('Ctrl Pts',(17.264575895997,17.1147192929918,-16.1110674280038));
#46629=CARTESIAN_POINT('Ctrl Pts',(17.1957120107061,17.1629906206834,-16.1152429921954));
#46630=CARTESIAN_POINT('Ctrl Pts',(17.1292788382185,17.2146240223491,-16.1194185563871));
#46631=CARTESIAN_POINT('Ctrl Pts',(17.0656083164572,17.2693333987821,-16.1235941205788));
#46632=CARTESIAN_POINT('Ctrl Pts',(16.9987219480042,17.3268060157593,-16.1279805825913));
#46633=CARTESIAN_POINT('Ctrl Pts',(16.9348850702689,17.3876731058188,-16.1323670446039));
#46634=CARTESIAN_POINT('Ctrl Pts',(16.8744375629656,17.4515604464004,-16.1367535066164));
#46635=CARTESIAN_POINT('Ctrl Pts',(16.8139900556624,17.515447786982,-16.141139968629));
#46636=CARTESIAN_POINT('Ctrl Pts',(16.7569322374058,17.5823548872471,-16.1455264306415));
#46637=CARTESIAN_POINT('Ctrl Pts',(16.703552701499,17.6518708302357,-16.149912892654));
#46638=CARTESIAN_POINT('Ctrl Pts',(16.652554439824,17.7182856499019,-16.1541036735168));
#46639=CARTESIAN_POINT('Ctrl Pts',(16.6047208600205,17.7873320135743,-16.1582944543796));
#46640=CARTESIAN_POINT('Ctrl Pts',(16.5603345705064,17.8586765917043,-16.1624852352424));
#46641=CARTESIAN_POINT('Ctrl Pts',(16.5160108372518,17.9299206196422,-16.1666701097864));
#46642=CARTESIAN_POINT('Ctrl Pts',(16.4751249866853,18.0034560458725,-16.1708549843304));
#46643=CARTESIAN_POINT('Ctrl Pts',(16.4379187528239,18.0789174471946,-16.1750398588744));
#46644=CARTESIAN_POINT('Ctrl Pts',(16.4007539244062,18.15429487031,-16.1792200762261));
#46645=CARTESIAN_POINT('Ctrl Pts',(16.367260780246,18.2315936031771,-16.1834002935778));
#46646=CARTESIAN_POINT('Ctrl Pts',(16.3376364602561,18.3104214163183,-16.1875805109295));
#46647=CARTESIAN_POINT('Ctrl Pts',(16.3080359860438,18.3891857778597,-16.1917573634602));
#46648=CARTESIAN_POINT('Ctrl Pts',(16.2822983085872,18.4694763469326,-16.1959342159909));
#46649=CARTESIAN_POINT('Ctrl Pts',(16.2605729619713,18.5508797931071,-16.2001110685216));
#46650=CARTESIAN_POINT('Ctrl Pts',(16.238858101653,18.632243947813,-16.2042859049869));
#46651=CARTESIAN_POINT('Ctrl Pts',(16.2211518401951,18.7147194701818,-16.2084607414522));
#46652=CARTESIAN_POINT('Ctrl Pts',(16.2075538451844,18.7978779516685,-16.2126355779176));
#46653=CARTESIAN_POINT('Ctrl Pts',(16.1939550163504,18.8810415323988,-16.2168106703821));
#46654=CARTESIAN_POINT('Ctrl Pts',(16.1844650395064,18.964887705472,-16.2209857628467));
#46655=CARTESIAN_POINT('Ctrl Pts',(16.1791322578277,19.048978951962,-16.2251608553112));
#46656=CARTESIAN_POINT('Ctrl Pts',(16.1756711337435,19.1035565169223,-16.227870606798));
#46657=CARTESIAN_POINT('Ctrl Pts',(16.1739601228212,19.158237148325,-16.2305803582847));
#46658=CARTESIAN_POINT('Ctrl Pts',(16.174000705501,19.2129005695108,-16.2332901097715));
#46659=CARTESIAN_POINT('Ctrl Pts',(16.1740007055014,19.2129005700936,-16.2332901098004));
#46660=CARTESIAN_POINT('Ctrl Pts',(16.1740727513108,19.3099436741144,-16.2381006886061));
#46661=CARTESIAN_POINT('Ctrl Pts',(16.1796667621362,19.4067618611662,-16.2429112674118));
#46662=CARTESIAN_POINT('Ctrl Pts',(16.1906824963736,19.5027808693996,-16.2477218462175));
#46663=CARTESIAN_POINT('Ctrl Pts',(16.201890345519,19.6004744535201,-16.2526163217372));
#46664=CARTESIAN_POINT('Ctrl Pts',(16.218710639996,19.6973405506009,-16.2575107972568));
#46665=CARTESIAN_POINT('Ctrl Pts',(16.2409867483461,19.7927945746377,-16.2624052727765));
#46666=CARTESIAN_POINT('Ctrl Pts',(16.2632628566961,19.8882485986746,-16.2672997482961));
#46667=CARTESIAN_POINT('Ctrl Pts',(16.2909946214077,19.9822904288897,-16.2721942238158));
#46668=CARTESIAN_POINT('Ctrl Pts',(16.3239764935689,20.074357804418,-16.2770886993355));
#46669=CARTESIAN_POINT('Ctrl Pts',(16.3521750361989,20.1530727360925,-16.2812733337285));
#46670=CARTESIAN_POINT('Ctrl Pts',(16.3842865295797,20.2305511910394,-16.2854579681216));
#46671=CARTESIAN_POINT('Ctrl Pts',(16.4201827606335,20.3063765484118,-16.2896426025146));
#46672=CARTESIAN_POINT('Ctrl Pts',(16.4560278978456,20.3820939777733,-16.2938212805986));
#46673=CARTESIAN_POINT('Ctrl Pts',(16.4956468770878,20.4561625710813,-16.2979999586825));
#46674=CARTESIAN_POINT('Ctrl Pts',(16.5388624466769,20.5281830252439,-16.3021786367664));
#46675=CARTESIAN_POINT('Ctrl Pts',(16.5828526242924,20.6014943942872,-16.3064322146519));
#46676=CARTESIAN_POINT('Ctrl Pts',(16.6305694356436,20.6726830222909,-16.3106857925373));
#46677=CARTESIAN_POINT('Ctrl Pts',(16.6817755898824,20.7413512572339,-16.3149393704228));
#46678=CARTESIAN_POINT('Ctrl Pts',(16.7319890129006,20.8086882244474,-16.3191104844007));
#46679=CARTESIAN_POINT('Ctrl Pts',(16.7855574030483,20.8736012662212,-16.3232815983787));
#46680=CARTESIAN_POINT('Ctrl Pts',(16.8422127801055,20.9357437823178,-16.3274527123566));
#46681=CARTESIAN_POINT('Ctrl Pts',(16.8988491459038,20.997865445893,-16.331622426677));
#46682=CARTESIAN_POINT('Ctrl Pts',(16.9585701316818,21.0572180904717,-16.3357921409973));
#46683=CARTESIAN_POINT('Ctrl Pts',(17.0210683042879,21.1134891605013,-16.3399618553177));
#46684=CARTESIAN_POINT('Ctrl Pts',(17.0835642529408,21.1697582281647,-16.3441314212618));
#46685=CARTESIAN_POINT('Ctrl Pts',(17.1488368494857,21.2229456321214,-16.3483009872058));
#46686=CARTESIAN_POINT('Ctrl Pts',(17.2165437463578,21.2727775142537,-16.3524705531499));
#46687=CARTESIAN_POINT('Ctrl Pts',(17.2866311341984,21.3243614238875,-16.3567867158888));
#46688=CARTESIAN_POINT('Ctrl Pts',(17.3593267625536,21.3723491485032,-16.3611028786277));
#46689=CARTESIAN_POINT('Ctrl Pts',(17.4342176396321,21.4164853923063,-16.3654190413666));
#46690=CARTESIAN_POINT('Ctrl Pts',(17.5066689542669,21.4591839026099,-16.3695946055583));
#46691=CARTESIAN_POINT('Ctrl Pts',(17.5811742544608,21.4982778256331,-16.37377016975));
#46692=CARTESIAN_POINT('Ctrl Pts',(17.6573356824291,21.533583464005,-16.3779457339417));
#46693=CARTESIAN_POINT('Ctrl Pts',(17.7373438430675,21.5706723062399,-16.3823321959542));
#46694=CARTESIAN_POINT('Ctrl Pts',(17.8191792885613,21.6035798961265,-16.3867186579667));
#46695=CARTESIAN_POINT('Ctrl Pts',(17.9023606575271,21.6321517928563,-16.3911051199793));
#46696=CARTESIAN_POINT('Ctrl Pts',(17.985542026493,21.6607236895861,-16.3954915819918));
#46697=CARTESIAN_POINT('Ctrl Pts',(18.0700687402226,21.6849598063577,-16.3998780440043));
#46698=CARTESIAN_POINT('Ctrl Pts',(18.1554472698608,21.7047675790756,-16.4042645060169));
#46699=CARTESIAN_POINT('Ctrl Pts',(18.2369040239201,21.7236655019793,-16.4084494803759));
#46700=CARTESIAN_POINT('Ctrl Pts',(18.3194392781939,21.7386033270985,-16.4126344547349));
#46701=CARTESIAN_POINT('Ctrl Pts',(18.4026332182035,21.7494633256996,-16.4168194290939));
#46702=CARTESIAN_POINT('Ctrl Pts',(18.4856850454026,21.7603047731307,-16.4209972546333));
#46703=CARTESIAN_POINT('Ctrl Pts',(18.5693928687513,21.7670821859801,-16.4251750801727));
#46704=CARTESIAN_POINT('Ctrl Pts',(18.6533252588855,21.7697285096598,-16.4293529057122));
#46705=CARTESIAN_POINT('Ctrl Pts',(18.7371760689815,21.7723722611838,-16.4335266705169));
#46706=CARTESIAN_POINT('Ctrl Pts',(18.821250555471,21.7708928806735,-16.4377004353216));
#46707=CARTESIAN_POINT('Ctrl Pts',(18.9051115090561,21.7652750148464,-16.4418742001264));
#46708=CARTESIAN_POINT('Ctrl Pts',(18.9889161108075,21.7596609240425,-16.4460451602969));
#46709=CARTESIAN_POINT('Ctrl Pts',(19.0725070069924,21.7499139014393,-16.4502161204674));
#46710=CARTESIAN_POINT('Ctrl Pts',(19.1554476929899,21.736070660808,-16.4543870806379));
#46711=CARTESIAN_POINT('Ctrl Pts',(19.238357526517,21.7222325696177,-16.4585564892849));
#46712=CARTESIAN_POINT('Ctrl Pts',(19.3206171772896,21.7043013640799,-16.4627258979319));
#46713=CARTESIAN_POINT('Ctrl Pts',(19.4017973253961,21.682365357893,-16.4668953065789));
#46714=CARTESIAN_POINT('Ctrl Pts',(19.4830102717192,21.6604204891714,-16.4710663997407));
#46715=CARTESIAN_POINT('Ctrl Pts',(19.5631423969819,21.6344676983522,-16.4752374929026));
#46716=CARTESIAN_POINT('Ctrl Pts',(19.6417773433648,21.6046458165053,-16.4794085860645));
#46717=CARTESIAN_POINT('Ctrl Pts',(19.7204244341702,21.5748193289513,-16.4835803234122));
#46718=CARTESIAN_POINT('Ctrl Pts',(19.7975734594199,21.5411227351377,-16.4877520607599));
#46719=CARTESIAN_POINT('Ctrl Pts',(19.8728278889751,21.5037431254488,-16.4919237981076));
#46720=CARTESIAN_POINT('Ctrl Pts',(19.9481771492335,21.4663164124239,-16.4961007924055));
#46721=CARTESIAN_POINT('Ctrl Pts',(20.0216266360793,21.425197626564,-16.5002777867034));
#46722=CARTESIAN_POINT('Ctrl Pts',(20.0928045893704,21.3806198026166,-16.5044547810012));
#46723=CARTESIAN_POINT('Ctrl Pts',(20.1619637761317,21.337306305821,-16.5085133063646));
#46724=CARTESIAN_POINT('Ctrl Pts',(20.2289782723143,21.2907276477199,-16.5125718317281));
#46725=CARTESIAN_POINT('Ctrl Pts',(20.2935358855687,21.2411349269503,-16.5166303570915));
#46726=CARTESIAN_POINT('',(16.1740005630998,19.2093020392336,-16.1667098902285));
#46727=CARTESIAN_POINT('Ctrl Pts',(16.1740005630998,19.2093020392336,-16.1667098902285));
#46728=CARTESIAN_POINT('Ctrl Pts',(16.1739457994085,19.2918687402816,-16.1708335669039));
#46729=CARTESIAN_POINT('Ctrl Pts',(16.1778897355288,19.3745927743499,-16.1749572435793));
#46730=CARTESIAN_POINT('Ctrl Pts',(16.185851592152,19.4570481489095,-16.1790809202548));
#46731=CARTESIAN_POINT('Ctrl Pts',(16.193849980064,19.5398818524496,-16.1832235175451));
#46732=CARTESIAN_POINT('Ctrl Pts',(16.2059033176551,19.6224439445466,-16.1873661148355));
#46733=CARTESIAN_POINT('Ctrl Pts',(16.2219780566694,19.7043008779901,-16.1915087121259));
#46734=CARTESIAN_POINT('Ctrl Pts',(16.23794569149,19.7856124078128,-16.1956237077524));
#46735=CARTESIAN_POINT('Ctrl Pts',(16.2578812222445,19.8662276743518,-16.1997387033789));
#46736=CARTESIAN_POINT('Ctrl Pts',(16.2816998746989,19.9457272251988,-16.2038536990054));
#46737=CARTESIAN_POINT('Ctrl Pts',(16.3055083094403,20.0251926723702,-16.2079669293832));
#46738=CARTESIAN_POINT('Ctrl Pts',(16.33319642467,20.1035429002386,-16.2120801597611));
#46739=CARTESIAN_POINT('Ctrl Pts',(16.3646289972004,20.1803714721883,-16.2161933901389));
#46740=CARTESIAN_POINT('Ctrl Pts',(16.3960581246075,20.2571916234494,-16.2203061696919));
#46741=CARTESIAN_POINT('Ctrl Pts',(16.4312307139715,20.3324900117992,-16.2244189492448));
#46742=CARTESIAN_POINT('Ctrl Pts',(16.469963164482,20.405879578626,-16.2285317287978));
#46743=CARTESIAN_POINT('Ctrl Pts',(16.5091807554344,20.48018838104,-16.2326960226666));
#46744=CARTESIAN_POINT('Ctrl Pts',(16.5520477937182,20.552539761255,-16.2368603165354));
#46745=CARTESIAN_POINT('Ctrl Pts',(16.5983263505016,20.6225587351713,-16.2410246104042));
#46746=CARTESIAN_POINT('Ctrl Pts',(16.6440925485817,20.6918025157112,-16.2451428005837));
#46747=CARTESIAN_POINT('Ctrl Pts',(16.6931947649456,20.7587649302322,-16.2492609907631));
#46748=CARTESIAN_POINT('Ctrl Pts',(16.7453611252724,20.8231152024351,-16.2533791809425));
#46749=CARTESIAN_POINT('Ctrl Pts',(16.7984034996618,20.8885460894828,-16.257566526656));
#46750=CARTESIAN_POINT('Ctrl Pts',(16.8546135316783,20.9512759179513,-16.2617538723695));
#46751=CARTESIAN_POINT('Ctrl Pts',(16.9136665630956,21.010996160687,-16.265941218083));
#46752=CARTESIAN_POINT('Ctrl Pts',(16.972719594513,21.0707164034227,-16.2701285637965));
#46753=CARTESIAN_POINT('Ctrl Pts',(17.0346152026565,21.1274267716985,-16.2743159095101));
#46754=CARTESIAN_POINT('Ctrl Pts',(17.0989955289249,21.1808630357374,-16.2785032552236));
#46755=CARTESIAN_POINT('Ctrl Pts',(17.1633341687151,21.2342646996152,-16.2826878896166));
#46756=CARTESIAN_POINT('Ctrl Pts',(17.2304115572045,21.2846103343966,-16.2868725240096));
#46757=CARTESIAN_POINT('Ctrl Pts',(17.29990527078,21.3316065895454,-16.2910571584027));
#46758=CARTESIAN_POINT('Ctrl Pts',(17.3693000686558,21.378535951342,-16.2952358364866));
#46759=CARTESIAN_POINT('Ctrl Pts',(17.4411039821925,21.4221251476138,-16.2994145145706));
#46760=CARTESIAN_POINT('Ctrl Pts',(17.5149611920068,21.4621206952553,-16.3035931926545));
#46761=CARTESIAN_POINT('Ctrl Pts',(17.5901422392269,21.5028331343439,-16.30784677054));
#46762=CARTESIAN_POINT('Ctrl Pts',(17.6674505464319,21.5398215173808,-16.3121003484254));
#46763=CARTESIAN_POINT('Ctrl Pts',(17.7464794551571,21.5728643427414,-16.3163539263108));
#46764=CARTESIAN_POINT('Ctrl Pts',(17.8239762342744,21.6052665684546,-16.3205250402888));
#46765=CARTESIAN_POINT('Ctrl Pts',(17.9031270518499,21.6338746703221,-16.3246961542667));
#46766=CARTESIAN_POINT('Ctrl Pts',(17.983524818815,21.6585267112792,-16.3288672682447));
#46767=CARTESIAN_POINT('Ctrl Pts',(18.0638956075329,21.6831704800059,-16.3330369825651));
#46768=CARTESIAN_POINT('Ctrl Pts',(18.1455120751846,21.7038606894987,-16.3372066968854));
#46769=CARTESIAN_POINT('Ctrl Pts',(18.2279505020329,21.7204847888774,-16.3413764112058));
#46770=CARTESIAN_POINT('Ctrl Pts',(18.3103859953682,21.7371082966994,-16.3455459771499));
#46771=CARTESIAN_POINT('Ctrl Pts',(18.3936429386223,21.7496658919856,-16.3497155430939));
#46772=CARTESIAN_POINT('Ctrl Pts',(18.4772872562561,21.758096104822,-16.353885109038));
#46773=CARTESIAN_POINT('Ctrl Pts',(18.5638724049115,21.7668227135419,-16.3582012717769));
#46774=CARTESIAN_POINT('Ctrl Pts',(18.6508721501767,21.7711262492444,-16.3625174345158));
#46775=CARTESIAN_POINT('Ctrl Pts',(18.7378010569183,21.7709971781169,-16.3668335972547));
#46776=CARTESIAN_POINT('Ctrl Pts',(18.821898263666,21.7708723114677,-16.3710091614464));
#46777=CARTESIAN_POINT('Ctrl Pts',(18.9059287081103,21.7665992585964,-16.3751847256381));
#46778=CARTESIAN_POINT('Ctrl Pts',(18.9894564259431,21.7582224116563,-16.3793602898298));
#46779=CARTESIAN_POINT('Ctrl Pts',(19.0772029302354,21.7494224700914,-16.3837467518423));
#46780=CARTESIAN_POINT('Ctrl Pts',(19.1643940106309,21.7360933624401,-16.3881332138549));
#46781=CARTESIAN_POINT('Ctrl Pts',(19.2505367177895,21.7183471676605,-16.3925196758674));
#46782=CARTESIAN_POINT('Ctrl Pts',(19.3366794249481,21.700600972881,-16.3969061378799));
#46783=CARTESIAN_POINT('Ctrl Pts',(19.4217732165569,21.6784379108237,-16.4012925998925));
#46784=CARTESIAN_POINT('Ctrl Pts',(19.5053461655911,21.652029514944,-16.405679061905));
#46785=CARTESIAN_POINT('Ctrl Pts',(19.5850559562968,21.6268418467719,-16.4098627597761));
#46786=CARTESIAN_POINT('Ctrl Pts',(19.6636790298746,21.5976989266396,-16.4140464576472));
#46787=CARTESIAN_POINT('Ctrl Pts',(19.7407944846494,21.5647129956049,-16.4182301555184));
#46788=CARTESIAN_POINT('Ctrl Pts',(19.817813812667,21.5317681825354,-16.422408638283));
#46789=CARTESIAN_POINT('Ctrl Pts',(19.8933288322741,21.4949900441864,-16.4265871210476));
#46790=CARTESIAN_POINT('Ctrl Pts',(19.9669338586835,21.4545405278514,-16.4307656038122));
#46791=CARTESIAN_POINT('Ctrl Pts',(20.0404561874615,21.4141364578583,-16.4349393919161));
#46792=CARTESIAN_POINT('Ctrl Pts',(20.1120723866535,21.3700694275403,-16.43911318002));
#46793=CARTESIAN_POINT('Ctrl Pts',(20.1813982979661,21.3225487602812,-16.4432869681239));
#46794=CARTESIAN_POINT('Ctrl Pts',(20.2194886441686,21.2964390614196,-16.4455802092922));
#46795=CARTESIAN_POINT('Ctrl Pts',(20.2568879835979,21.2692875967535,-16.4478734504605));
#46796=CARTESIAN_POINT('Ctrl Pts',(20.2935358855687,21.2411349269503,-16.4501666916289));
#46797=CARTESIAN_POINT('Ctrl Pts',(20.2958871626529,21.2441650537926,-15.6501589834813));
#46798=CARTESIAN_POINT('Ctrl Pts',(20.9266956913523,20.7545799070163,-15.6900393318202));
#46799=CARTESIAN_POINT('Ctrl Pts',(21.7315666544893,19.0879531984753,-15.7723116157195));
#46800=CARTESIAN_POINT('Ctrl Pts',(20.3102572494442,16.6266809282313,-15.8969758351793));
#46801=CARTESIAN_POINT('Ctrl Pts',(17.4141947910433,16.4867742032747,-16.0241516418607));
#46802=CARTESIAN_POINT('Ctrl Pts',(16.2227678179363,18.1548349051303,-16.1140629935438));
#46803=CARTESIAN_POINT('Ctrl Pts',(16.1704458861955,19.106523168223,-16.1615824096664));
#46804=CARTESIAN_POINT('Ctrl Pts',(16.1712324881214,19.2093002032634,-16.1667098902285));
#46805=CARTESIAN_POINT('Origin',(18.734,19.211,1.76670989022852));
#46806=CARTESIAN_POINT('',(20.2935358855687,21.2411349269503,-14.8500370294445));
#46807=CARTESIAN_POINT('',(20.2935358855687,21.2411349269503,-14.9167585822245));
#46808=CARTESIAN_POINT('',(20.2935358855687,21.2411349269503,1.76670989022852));
#46809=CARTESIAN_POINT('',(16.174000571626,19.2092892327452,-15.4332901097416));
#46810=CARTESIAN_POINT('Ctrl Pts',(20.2935358855687,21.2411349269503,-14.9167585822245));
#46811=CARTESIAN_POINT('Ctrl Pts',(20.3601520146462,21.1899608682831,-14.9209295765852));
#46812=CARTESIAN_POINT('Ctrl Pts',(20.4242947432533,21.1354675703399,-14.9251005709459));
#46813=CARTESIAN_POINT('Ctrl Pts',(20.4856216544896,21.0779283809303,-14.9292715653066));
#46814=CARTESIAN_POINT('Ctrl Pts',(20.5469290937748,21.0204074608296,-14.9334412353319));
#46815=CARTESIAN_POINT('Ctrl Pts',(20.6054221561177,20.9598428845434,-14.9376109053571));
#46816=CARTESIAN_POINT('Ctrl Pts',(20.6607930923822,20.8965469080237,-14.9417805753824));
#46817=CARTESIAN_POINT('Ctrl Pts',(20.7161630576809,20.8332520414406,-14.9459501722898));
#46818=CARTESIAN_POINT('Ctrl Pts',(20.7684107036615,20.7672262168081,-14.9501197691972));
#46819=CARTESIAN_POINT('Ctrl Pts',(20.8172675280852,20.6988159854048,-14.9542893661046));
#46820=CARTESIAN_POINT('Ctrl Pts',(20.86710676209,20.6290301658912,-14.9585428049726));
#46821=CARTESIAN_POINT('Ctrl Pts',(20.9134170181936,20.5567633970815,-14.9627962438407));
#46822=CARTESIAN_POINT('Ctrl Pts',(20.9559598075288,20.482414414629,-14.9670496827087));
#46823=CARTESIAN_POINT('Ctrl Pts',(20.9977248080393,20.4094247179354,-14.9712253580528));
#46824=CARTESIAN_POINT('Ctrl Pts',(21.0358587895228,20.3344287511086,-14.9754010333968));
#46825=CARTESIAN_POINT('Ctrl Pts',(21.0701835569614,20.2578268186205,-14.9795767087409));
#46826=CARTESIAN_POINT('Ctrl Pts',(21.1054671686548,20.1790850515945,-14.9838690293709));
#46827=CARTESIAN_POINT('Ctrl Pts',(21.1367253886224,20.0986467474965,-14.988161350001));
#46828=CARTESIAN_POINT('Ctrl Pts',(21.1638191362431,20.0169646178008,-14.992453670631));
#46829=CARTESIAN_POINT('Ctrl Pts',(21.1909128838638,19.9352824881052,-14.996745991261));
#46830=CARTESIAN_POINT('Ctrl Pts',(21.2138420873009,19.8523570528488,-15.0010383118911));
#46831=CARTESIAN_POINT('Ctrl Pts',(21.2325245180281,19.7686515334979,-15.0053306325211));
#46832=CARTESIAN_POINT('Ctrl Pts',(21.2507382417699,19.6870460279088,-15.0095152669142));
#46833=CARTESIAN_POINT('Ctrl Pts',(21.2649836214983,19.6043953888037,-15.0136999013072));
#46834=CARTESIAN_POINT('Ctrl Pts',(21.2751464736302,19.5211202985241,-15.0178845357003));
#46835=CARTESIAN_POINT('Ctrl Pts',(21.2852948602001,19.437963740028,-15.0220632137842));
#46836=CARTESIAN_POINT('Ctrl Pts',(21.2913722063419,19.3541849485906,-15.0262418918682));
#46837=CARTESIAN_POINT('Ctrl Pts',(21.2933150345072,19.2702161645608,-15.0304205699521));
#46838=CARTESIAN_POINT('Ctrl Pts',(21.2952926864712,19.1847423004247,-15.0346741478376));
#46839=CARTESIAN_POINT('Ctrl Pts',(21.2929860350543,19.0990720360279,-15.038927725723));
#46840=CARTESIAN_POINT('Ctrl Pts',(21.2863832385264,19.0136682902077,-15.0431813036084));
#46841=CARTESIAN_POINT('Ctrl Pts',(21.2799084500934,18.929920262652,-15.0473524175864));
#46842=CARTESIAN_POINT('Ctrl Pts',(21.2693026454396,18.8464289917131,-15.0515235315643));
#46843=CARTESIAN_POINT('Ctrl Pts',(21.2546071988875,18.7636306348034,-15.0556946455423));
#46844=CARTESIAN_POINT('Ctrl Pts',(21.2399166835344,18.6808600616818,-15.0598643598627));
#46845=CARTESIAN_POINT('Ctrl Pts',(21.2211393320556,18.5987823933899,-15.0640340741831));
#46846=CARTESIAN_POINT('Ctrl Pts',(21.1983680574963,18.5178260844552,-15.0682037885034));
#46847=CARTESIAN_POINT('Ctrl Pts',(21.1755975932368,18.4368726562935,-15.0723733544475));
#46848=CARTESIAN_POINT('Ctrl Pts',(21.1488336138536,18.357040950769,-15.0765429203915));
#46849=CARTESIAN_POINT('Ctrl Pts',(21.1182192201023,18.2787453617736,-15.0807124863356));
#46850=CARTESIAN_POINT('Ctrl Pts',(21.0865284620337,18.1976969964573,-15.0850286490745));
#46851=CARTESIAN_POINT('Ctrl Pts',(21.0507116827587,18.1182952684024,-15.0893448118134));
#46852=CARTESIAN_POINT('Ctrl Pts',(21.0109816181364,18.0409766196058,-15.0936609745523));
#46853=CARTESIAN_POINT('Ctrl Pts',(20.9725457561902,17.9661766176612,-15.097836538744));
#46854=CARTESIAN_POINT('Ctrl Pts',(20.9304479207722,17.8933264506918,-15.1020121029357));
#46855=CARTESIAN_POINT('Ctrl Pts',(20.884926303708,17.8227939504464,-15.1061876671274));
#46856=CARTESIAN_POINT('Ctrl Pts',(20.8371054979832,17.7486990212888,-15.1105741291399));
#46857=CARTESIAN_POINT('Ctrl Pts',(20.7855062921192,17.6771625161638,-15.1149605911524));
#46858=CARTESIAN_POINT('Ctrl Pts',(20.7304530967375,17.6085721443612,-15.119347053165));
#46859=CARTESIAN_POINT('Ctrl Pts',(20.6753999013558,17.5399817725586,-15.1237335151775));
#46860=CARTESIAN_POINT('Ctrl Pts',(20.616893159293,17.4743379166139,-15.12811997719));
#46861=CARTESIAN_POINT('Ctrl Pts',(20.5553006227462,17.4119824788001,-15.1325064392026));
#46862=CARTESIAN_POINT('Ctrl Pts',(20.496542050108,17.352496107113,-15.1366910735956));
#46863=CARTESIAN_POINT('Ctrl Pts',(20.4347566962297,17.2957807737874,-15.1408757079887));
#46864=CARTESIAN_POINT('Ctrl Pts',(20.3702364829786,17.2421601965193,-15.1450603423817));
#46865=CARTESIAN_POINT('Ctrl Pts',(20.3058081062651,17.1886159415061,-15.1492390204657));
#46866=CARTESIAN_POINT('Ctrl Pts',(20.2386529531481,17.1381579843472,-15.1534176985496));
#46867=CARTESIAN_POINT('Ctrl Pts',(20.1691001101646,17.0910736631181,-15.1575963766336));
#46868=CARTESIAN_POINT('Ctrl Pts',(20.0983005824573,17.0431453892698,-15.161849954519));
#46869=CARTESIAN_POINT('Ctrl Pts',(20.0250169010501,16.9987132288229,-15.1661035324044));
#46870=CARTESIAN_POINT('Ctrl Pts',(19.9496318977225,16.9580377079854,-15.1703571102899));
#46871=CARTESIAN_POINT('Ctrl Pts',(19.8757083797862,16.9181507614911,-15.1745282242678));
#46872=CARTESIAN_POINT('Ctrl Pts',(19.7997647128027,16.8818763233781,-15.1786993382458));
#46873=CARTESIAN_POINT('Ctrl Pts',(19.7221900312683,16.8494156881233,-15.1828704522237));
#46874=CARTESIAN_POINT('Ctrl Pts',(19.6446413806673,16.8169659453482,-15.1870401665441));
#46875=CARTESIAN_POINT('Ctrl Pts',(19.5654632264915,16.7883276412413,-15.1912098808645));
#46876=CARTESIAN_POINT('Ctrl Pts',(19.4850661232635,16.7636545649447,-15.1953795951849));
#46877=CARTESIAN_POINT('Ctrl Pts',(19.4046718809096,16.7389823666222,-15.1995491611289));
#46878=CARTESIAN_POINT('Ctrl Pts',(19.3230592157838,16.7182752497195,-15.2037187270729));
#46879=CARTESIAN_POINT('Ctrl Pts',(19.2406540252948,16.7016371927016,-15.207888293017));
#46880=CARTESIAN_POINT('Ctrl Pts',(19.1553515699658,16.6844141621241,-15.2122044557559));
#46881=CARTESIAN_POINT('Ctrl Pts',(19.0692003389648,16.6715517559429,-15.2165206184948));
#46882=CARTESIAN_POINT('Ctrl Pts',(18.9826824608285,16.6631073347418,-15.2208367812337));
#46883=CARTESIAN_POINT('Ctrl Pts',(18.8989828934724,16.6549379896732,-15.2250123454254));
#46884=CARTESIAN_POINT('Ctrl Pts',(18.8149406719769,16.650903193465,-15.2291879096171));
#46885=CARTESIAN_POINT('Ctrl Pts',(18.7309940133495,16.6510017648357,-15.2333634738088));
#46886=CARTESIAN_POINT('Ctrl Pts',(18.6428074085591,16.6511053148121,-15.2377499358213));
#46887=CARTESIAN_POINT('Ctrl Pts',(18.5547268571684,16.6557707277653,-15.2421363978338));
#46888=CARTESIAN_POINT('Ctrl Pts',(18.4672539586503,16.6649350853868,-15.2465228598464));
#46889=CARTESIAN_POINT('Ctrl Pts',(18.3797810601322,16.6740994430083,-15.2509093218589));
#46890=CARTESIAN_POINT('Ctrl Pts',(18.2929163758375,16.6877625800018,-15.2552957838715));
#46891=CARTESIAN_POINT('Ctrl Pts',(18.2071464487601,16.7058003401833,-15.259682245884));
#46892=CARTESIAN_POINT('Ctrl Pts',(18.125322923169,16.7230081562804,-15.2638668802771));
#46893=CARTESIAN_POINT('Ctrl Pts',(18.0441910630359,16.74426092691,-15.2680515146701));
#46894=CARTESIAN_POINT('Ctrl Pts',(17.9641810754836,16.7694884142285,-15.2722361490632));
#46895=CARTESIAN_POINT('Ctrl Pts',(17.8842849722453,16.7946799933414,-15.2764148271471));
#46896=CARTESIAN_POINT('Ctrl Pts',(17.8055080047355,16.8238349143801,-15.2805935052311));
#46897=CARTESIAN_POINT('Ctrl Pts',(17.7282699071042,16.8568319982967,-15.284772183315));
#46898=CARTESIAN_POINT('Ctrl Pts',(17.6496473720828,16.8904205312279,-15.2890257612004));
#46899=CARTESIAN_POINT('Ctrl Pts',(17.5726198898781,16.92799022417,-15.2932793390859));
#46900=CARTESIAN_POINT('Ctrl Pts',(17.4976137413829,16.969360194076,-15.2975329169713));
#46901=CARTESIAN_POINT('Ctrl Pts',(17.4240617334388,17.0099281263886,-15.3017040309493));
#46902=CARTESIAN_POINT('Ctrl Pts',(17.3524538049873,17.0541500666244,-15.3058751449272));
#46903=CARTESIAN_POINT('Ctrl Pts',(17.2831698439506,17.1018077711367,-15.3100462589052));
#46904=CARTESIAN_POINT('Ctrl Pts',(17.213909131816,17.1494494836459,-15.3142159732255));
#46905=CARTESIAN_POINT('Ctrl Pts',(17.1469712170492,17.2005244102484,-15.3183856875459));
#46906=CARTESIAN_POINT('Ctrl Pts',(17.0827076373572,17.2547705827083,-15.3225554018663));
#46907=CARTESIAN_POINT('Ctrl Pts',(17.0184463444391,17.3090148248566,-15.3267249678103));
#46908=CARTESIAN_POINT('Ctrl Pts',(16.9568595483702,17.3664297911053,-15.3308945337544));
#46909=CARTESIAN_POINT('Ctrl Pts',(16.8982652087739,17.4267136507045,-15.3350640996984));
#46910=CARTESIAN_POINT('Ctrl Pts',(16.8376107644814,17.489117016439,-15.3393802624373));
#46911=CARTESIAN_POINT('Ctrl Pts',(16.7801634890495,17.5545943914719,-15.3436964251763));
#46912=CARTESIAN_POINT('Ctrl Pts',(16.7262325806842,17.6227714301985,-15.3480125879152));
#46913=CARTESIAN_POINT('Ctrl Pts',(16.6740584659863,17.6887276090595,-15.3521881521069));
#46914=CARTESIAN_POINT('Ctrl Pts',(16.6251753803868,17.7572098587058,-15.3563637162986));
#46915=CARTESIAN_POINT('Ctrl Pts',(16.5798195291696,17.8278490685782,-15.3605392804902));
#46916=CARTESIAN_POINT('Ctrl Pts',(16.5321728617309,17.9020560970123,-15.3649257425028));
#46917=CARTESIAN_POINT('Ctrl Pts',(16.488419403819,17.9786432012274,-15.3693122045153));
#46918=CARTESIAN_POINT('Ctrl Pts',(16.4487777573745,18.0571545589595,-15.3736986665278));
#46919=CARTESIAN_POINT('Ctrl Pts',(16.4091361109301,18.1356659166917,-15.3780851285404));
#46920=CARTESIAN_POINT('Ctrl Pts',(16.3736064408137,18.2161009664618,-15.3824715905529));
#46921=CARTESIAN_POINT('Ctrl Pts',(16.3423477078172,18.2979833992217,-15.3868580525655));
#46922=CARTESIAN_POINT('Ctrl Pts',(16.3083133302776,18.3871366489943,-15.3916340140293));
#46923=CARTESIAN_POINT('Ctrl Pts',(16.2792349760219,18.4782809296076,-15.396409975493));
#46924=CARTESIAN_POINT('Ctrl Pts',(16.2553188691388,18.5708907503302,-15.4011859369568));
#46925=CARTESIAN_POINT('Ctrl Pts',(16.2315006236311,18.6631216245767,-15.4059423558521));
#46926=CARTESIAN_POINT('Ctrl Pts',(16.2128025911618,18.756805887815,-15.4106987747473));
#46927=CARTESIAN_POINT('Ctrl Pts',(16.1993817363335,18.8514026453261,-15.4154551936426));
#46928=CARTESIAN_POINT('Ctrl Pts',(16.1860549755608,18.9453361818529,-15.4201782651283));
#46929=CARTESIAN_POINT('Ctrl Pts',(16.1779317634136,19.0401692636772,-15.4249013366139));
#46930=CARTESIAN_POINT('Ctrl Pts',(16.1751178968034,19.1353535728534,-15.4296244080995));
#46931=CARTESIAN_POINT('Ctrl Pts',(16.1743899245164,19.1599785991389,-15.4308463086469));
#46932=CARTESIAN_POINT('Ctrl Pts',(16.1740170525925,19.1846270439603,-15.4320682091943));
#46933=CARTESIAN_POINT('Ctrl Pts',(16.174000571626,19.2092892327452,-15.4332901097416));
#46934=CARTESIAN_POINT('Ctrl Pts',(16.1740005716256,19.2092892333484,-15.4332901097715));
#46935=CARTESIAN_POINT('Ctrl Pts',(16.1739440307447,19.2938972788889,-15.437482057942));
#46936=CARTESIAN_POINT('Ctrl Pts',(16.1780862675835,19.3785303101354,-15.4416740061124));
#46937=CARTESIAN_POINT('Ctrl Pts',(16.1864081330308,19.4627452667924,-15.4458659542829));
#46938=CARTESIAN_POINT('Ctrl Pts',(16.1947304086796,19.5469643745742,-15.4500581090829));
#46939=CARTESIAN_POINT('Ctrl Pts',(16.2072326772703,19.6307649161166,-15.4542502638829));
#46940=CARTESIAN_POINT('Ctrl Pts',(16.2238439368849,19.713709199047,-15.458442418683));
#46941=CARTESIAN_POINT('Ctrl Pts',(16.2404607969944,19.7966814466863,-15.4626359868702));
#46942=CARTESIAN_POINT('Ctrl Pts',(16.261189311038,19.8787964183332,-15.4668295550574));
#46943=CARTESIAN_POINT('Ctrl Pts',(16.2859076895266,19.9596281048698,-15.4710231232447));
#46944=CARTESIAN_POINT('Ctrl Pts',(16.3106584247115,20.0405656011923,-15.4752221808702));
#46945=CARTESIAN_POINT('Ctrl Pts',(16.3394093150967,20.1202160261802,-15.4794212384956));
#46946=CARTESIAN_POINT('Ctrl Pts',(16.3719892689075,20.1981703531832,-15.4836202961211));
#46947=CARTESIAN_POINT('Ctrl Pts',(16.4045936038559,20.2761830171373,-15.4878224961023));
#46948=CARTESIAN_POINT('Ctrl Pts',(16.4410325111314,20.3524966484666,-15.4920246960834));
#46949=CARTESIAN_POINT('Ctrl Pts',(16.4810885578785,20.426726134439,-15.4962268960645));
#46950=CARTESIAN_POINT('Ctrl Pts',(16.5212156880345,20.5010873479616,-15.5004365532643));
#46951=CARTESIAN_POINT('Ctrl Pts',(16.5649725361191,20.5733566470847,-15.5046462104641));
#46952=CARTESIAN_POINT('Ctrl Pts',(16.6120981192869,20.6431775059769,-15.5088558676639));
#46953=CARTESIAN_POINT('Ctrl Pts',(16.6314200308982,20.6718046841136,-15.5105818648583));
#46954=CARTESIAN_POINT('Ctrl Pts',(16.6513077816385,20.700020648932,-15.5123078620526));
#46955=CARTESIAN_POINT('Ctrl Pts',(16.6717415022698,20.7278025212728,-15.5140338592469));
#46956=CARTESIAN_POINT('Ctrl Pts',(16.7212825156696,20.7951589334866,-15.5182184936399));
#46957=CARTESIAN_POINT('Ctrl Pts',(16.7742191330187,20.8602110167103,-15.522403128033));
#46958=CARTESIAN_POINT('Ctrl Pts',(16.8303093008605,20.9225962497066,-15.526587762426));
#46959=CARTESIAN_POINT('Ctrl Pts',(16.8863196312909,20.9848926850454,-15.53076644051));
#46960=CARTESIAN_POINT('Ctrl Pts',(16.9454742913218,21.044529470903,-15.5349451185939));
#46961=CARTESIAN_POINT('Ctrl Pts',(17.0074891937054,21.1011747103768,-15.5391237966779));
#46962=CARTESIAN_POINT('Ctrl Pts',(17.0706156686449,21.1588352750579,-15.5433773745633));
#46963=CARTESIAN_POINT('Ctrl Pts',(17.1367056485331,21.2133956031449,-15.5476309524487));
#46964=CARTESIAN_POINT('Ctrl Pts',(17.2054179892121,21.2645425577026,-15.5518845303342));
#46965=CARTESIAN_POINT('Ctrl Pts',(17.2727982070859,21.314697928741,-15.5560556443121));
#46966=CARTESIAN_POINT('Ctrl Pts',(17.3426996279385,21.3615708076596,-15.5602267582901));
#46967=CARTESIAN_POINT('Ctrl Pts',(17.4147663076934,21.4049057557432,-15.564397872268));
#46968=CARTESIAN_POINT('Ctrl Pts',(17.4868088047781,21.4482261623665,-15.5685675865884));
#46969=CARTESIAN_POINT('Ctrl Pts',(17.561014723861,21.4880107590573,-15.5727373009088));
#46970=CARTESIAN_POINT('Ctrl Pts',(17.6370000578042,21.5240480165406,-15.5769070152292));
#46971=CARTESIAN_POINT('Ctrl Pts',(17.7129826878631,21.5600839916636,-15.5810765811732));
#46972=CARTESIAN_POINT('Ctrl Pts',(17.7907441908666,21.5923726963449,-15.5852461471172));
#46973=CARTESIAN_POINT('Ctrl Pts',(17.8698781766135,21.6207496704735,-15.5894157130613));
#46974=CARTESIAN_POINT('Ctrl Pts',(17.951794415677,21.6501243440057,-15.5937318758002));
#46975=CARTESIAN_POINT('Ctrl Pts',(18.0351809497172,21.6753069180702,-15.5980480385391));
#46976=CARTESIAN_POINT('Ctrl Pts',(18.119569008403,21.6961709310559,-15.602364201278));
#46977=CARTESIAN_POINT('Ctrl Pts',(18.2012081349532,21.7163553010131,-15.6065397654697));
#46978=CARTESIAN_POINT('Ctrl Pts',(18.2837840674898,21.7324980994093,-15.6107153296614));
#46979=CARTESIAN_POINT('Ctrl Pts',(18.3668630221883,21.7445371399534,-15.6148908938531));
#46980=CARTESIAN_POINT('Ctrl Pts',(18.4541380973871,21.7571842438152,-15.6192773558656));
#46981=CARTESIAN_POINT('Ctrl Pts',(18.5419677640929,21.7653020795901,-15.6236638178781));
#46982=CARTESIAN_POINT('Ctrl Pts',(18.6298465962985,21.7688803858854,-15.6280502798907));
#46983=CARTESIAN_POINT('Ctrl Pts',(18.7177254285041,21.7724586921808,-15.6324367419032));
#46984=CARTESIAN_POINT('Ctrl Pts',(18.8056528468587,21.771497551399,-15.6368232039158));
#46985=CARTESIAN_POINT('Ctrl Pts',(18.8931294701918,21.7660494734381,-15.6412096659283));
#46986=CARTESIAN_POINT('Ctrl Pts',(18.9765715593009,21.7608526678304,-15.6453938186788));
#46987=CARTESIAN_POINT('Ctrl Pts',(19.0599140713073,21.7515543524027,-15.6495779714293));
#46988=CARTESIAN_POINT('Ctrl Pts',(19.1427213148452,21.7381618244171,-15.6537621241798));
#46989=CARTESIAN_POINT('Ctrl Pts',(19.2254168838743,21.7247873577016,-15.6579406341486));
#46990=CARTESIAN_POINT('Ctrl Pts',(19.307578167734,21.7073297146533,-15.6621191441173));
#46991=CARTESIAN_POINT('Ctrl Pts',(19.3887723742193,21.6858481040176,-15.6662976540861));
#46992=CARTESIAN_POINT('Ctrl Pts',(19.4703186692208,21.6642733410653,-15.6704942836404));
#46993=CARTESIAN_POINT('Ctrl Pts',(19.5508890103775,21.6386396544188,-15.6746909131948));
#46994=CARTESIAN_POINT('Ctrl Pts',(19.6300531105458,21.6090593868963,-15.6788875427491));
#46995=CARTESIAN_POINT('Ctrl Pts',(19.708732915175,21.5796600800816,-15.6830584989368));
#46996=CARTESIAN_POINT('Ctrl Pts',(19.7860231996119,21.5463625042622,-15.6872294551245));
#46997=CARTESIAN_POINT('Ctrl Pts',(19.8615163104711,21.5093269936242,-15.6914004113121));
#46998=CARTESIAN_POINT('Ctrl Pts',(19.9377064421921,21.4719495375657,-15.6956098775498));
#46999=CARTESIAN_POINT('Ctrl Pts',(20.0120655910137,21.430764917828,-15.6998193437875));
#47000=CARTESIAN_POINT('Ctrl Pts',(20.0841966760578,21.3859871116773,-15.7040288100252));
#47001=CARTESIAN_POINT('Ctrl Pts',(20.1563277611019,21.3412093055266,-15.7082382762629));
#47002=CARTESIAN_POINT('Ctrl Pts',(20.2262303717876,21.2928385662724,-15.7124477425006));
#47003=CARTESIAN_POINT('Ctrl Pts',(20.2935358855687,21.2411349269503,-15.7166572087383));
#47004=CARTESIAN_POINT('',(16.1740008768645,19.213118854712,-15.3667098902285));
#47005=CARTESIAN_POINT('Ctrl Pts',(16.1723624648697,19.2131202107894,-15.3667098902285));
#47006=CARTESIAN_POINT('Ctrl Pts',(16.1710770500739,19.3573559412274,-15.3738974629702));
#47007=CARTESIAN_POINT('Ctrl Pts',(16.2478506686825,20.350918062683,-15.4234769712723));
#47008=CARTESIAN_POINT('Ctrl Pts',(17.5479306856132,21.9960550376254,-15.515448415135));
#47009=CARTESIAN_POINT('Ctrl Pts',(19.528832106138,21.8036795310292,-15.6027438734776));
#47010=CARTESIAN_POINT('Ctrl Pts',(20.2561600613117,21.2749981796243,-15.6476473962597));
#47011=CARTESIAN_POINT('Ctrl Pts',(20.2958871626529,21.2441650537926,-15.6501589834813));
#47012=CARTESIAN_POINT('Ctrl Pts',(20.2935358855687,21.2411349269503,-14.8500370294445));
#47013=CARTESIAN_POINT('Ctrl Pts',(20.3601765745563,21.1899420015267,-14.8542147192048));
#47014=CARTESIAN_POINT('Ctrl Pts',(20.424227826631,21.1355151814304,-14.8583924089651));
#47015=CARTESIAN_POINT('Ctrl Pts',(20.4853757374046,21.078159079037,-14.8625700987253));
#47016=CARTESIAN_POINT('Ctrl Pts',(20.5466225419779,21.0207102152913,-14.8667545450143));
#47017=CARTESIAN_POINT('Ctrl Pts',(20.6049563163785,20.9603229457015,-14.8709389913032));
#47018=CARTESIAN_POINT('Ctrl Pts',(20.6601019149597,20.8973366844105,-14.8751234375922));
#47019=CARTESIAN_POINT('Ctrl Pts',(20.6796325157998,20.8750292009606,-14.8766054189707));
#47020=CARTESIAN_POINT('Ctrl Pts',(20.6987636044015,20.8523959980119,-14.8780874003493));
#47021=CARTESIAN_POINT('Ctrl Pts',(20.7174842649081,20.8294530178111,-14.8795693817278));
#47022=CARTESIAN_POINT('Ctrl Pts',(20.770345333846,20.764669488533,-14.8837540161209));
#47023=CARTESIAN_POINT('Ctrl Pts',(20.8201275486196,20.6971728954314,-14.8879386505139));
#47024=CARTESIAN_POINT('Ctrl Pts',(20.8665402687069,20.6272881071108,-14.892123284907));
#47025=CARTESIAN_POINT('Ctrl Pts',(20.9128869260319,20.5575027911363,-14.8963019629909));
#47026=CARTESIAN_POINT('Ctrl Pts',(20.9558733628217,20.4853364119635,-14.9004806410749));
#47027=CARTESIAN_POINT('Ctrl Pts',(20.995249084218,20.4111468989766,-14.9046593191588));
#47028=CARTESIAN_POINT('Ctrl Pts',(21.0353305871215,20.3356275922885,-14.9089128970442));
#47029=CARTESIAN_POINT('Ctrl Pts',(21.0716703524657,20.2580122826047,-14.9131664749297));
#47030=CARTESIAN_POINT('Ctrl Pts',(21.1040502914401,20.1787094688203,-14.9174200528151));
#47031=CARTESIAN_POINT('Ctrl Pts',(21.1358024821133,20.1009440948279,-14.9215911667931));
#47032=CARTESIAN_POINT('Ctrl Pts',(21.1637468322871,20.0215565094717,-14.925762280771));
#47033=CARTESIAN_POINT('Ctrl Pts',(21.1877248192282,19.9409551434873,-14.929933394749));
#47034=CARTESIAN_POINT('Ctrl Pts',(21.2116947601242,19.8603808240696,-14.9341031090693));
#47035=CARTESIAN_POINT('Ctrl Pts',(21.2317008500142,19.7785939734878,-14.9382728233897));
#47036=CARTESIAN_POINT('Ctrl Pts',(21.2476340898708,19.6960192390405,-14.9424425377101));
#47037=CARTESIAN_POINT('Ctrl Pts',(21.2635667627543,19.6134474429566,-14.9466121036541));
#47038=CARTESIAN_POINT('Ctrl Pts',(21.2754267874401,19.5300882706129,-14.9507816695982));
#47039=CARTESIAN_POINT('Ctrl Pts',(21.2831563307876,19.4463762970337,-14.9549512355422));
#47040=CARTESIAN_POINT('Ctrl Pts',(21.2911576353439,19.3597211137333,-14.9592673982811));
#47041=CARTESIAN_POINT('Ctrl Pts',(21.2947325504218,19.2726883838097,-14.9635835610201));
#47042=CARTESIAN_POINT('Ctrl Pts',(21.2938756072079,19.1857636052079,-14.967899723759));
#47043=CARTESIAN_POINT('Ctrl Pts',(21.293046578829,19.1016703921262,-14.9720752879507));
#47044=CARTESIAN_POINT('Ctrl Pts',(21.2880700686645,19.017678672767,-14.9762508521424));
#47045=CARTESIAN_POINT('Ctrl Pts',(21.2789941177452,18.9342240244488,-14.980426416334));
#47046=CARTESIAN_POINT('Ctrl Pts',(21.269459762121,18.8465542802384,-14.9848128783466));
#47047=CARTESIAN_POINT('Ctrl Pts',(21.2554010498833,18.7594778642491,-14.9891993403591));
#47048=CARTESIAN_POINT('Ctrl Pts',(21.2369341836446,18.6734867700758,-14.9935858023717));
#47049=CARTESIAN_POINT('Ctrl Pts',(21.2184673174058,18.5874956759025,-14.9979722643842));
#47050=CARTESIAN_POINT('Ctrl Pts',(21.1955925215496,18.5025904439986,-15.0023587263968));
#47051=CARTESIAN_POINT('Ctrl Pts',(21.1684852750763,18.4192415485537,-15.0067451884093));
#47052=CARTESIAN_POINT('Ctrl Pts',(21.1426252731958,18.3397276593411,-15.0109298228024));
#47053=CARTESIAN_POINT('Ctrl Pts',(21.1128174886273,18.2613340692511,-15.0151144571954));
#47054=CARTESIAN_POINT('Ctrl Pts',(21.0791777662536,18.1844810061817,-15.0192990915885));
#47055=CARTESIAN_POINT('Ctrl Pts',(21.0455859258609,18.1077373339352,-15.0234777696724));
#47056=CARTESIAN_POINT('Ctrl Pts',(21.0081731644857,18.0325302510435,-15.0276564477564));
#47057=CARTESIAN_POINT('Ctrl Pts',(20.9671048559809,17.9592641244279,-15.0318351258403));
#47058=CARTESIAN_POINT('Ctrl Pts',(20.9253004275615,17.8846847551481,-15.0360887037257));
#47059=CARTESIAN_POINT('Ctrl Pts',(20.8797082607491,17.8121170683452,-15.0403422816112));
#47060=CARTESIAN_POINT('Ctrl Pts',(20.8305537911316,17.7419655548996,-15.0445958594966));
#47061=CARTESIAN_POINT('Ctrl Pts',(20.7823522768247,17.6731740654314,-15.0487669734745));
#47062=CARTESIAN_POINT('Ctrl Pts',(20.7307256276405,17.6067062949759,-15.0529380874525));
#47063=CARTESIAN_POINT('Ctrl Pts',(20.675931463843,17.5429166118756,-15.0571092014304));
#47064=CARTESIAN_POINT('Ctrl Pts',(20.6211556867563,17.4791483340195,-15.0612789157508));
#47065=CARTESIAN_POINT('Ctrl Pts',(20.5632148054787,17.4180567074447,-15.0654486300712));
#47066=CARTESIAN_POINT('Ctrl Pts',(20.5024068820801,17.3599632366126,-15.0696183443916));
#47067=CARTESIAN_POINT('Ctrl Pts',(20.4416011224884,17.3018718329955,-15.0737879103356));
#47068=CARTESIAN_POINT('Ctrl Pts',(20.3779288568417,17.2467786901665,-15.0779574762796));
#47069=CARTESIAN_POINT('Ctrl Pts',(20.3117241899802,17.1949676638627,-15.0821270422237));
#47070=CARTESIAN_POINT('Ctrl Pts',(20.2431918487043,17.1413350257899,-15.0864432049626));
#47071=CARTESIAN_POINT('Ctrl Pts',(20.1719461297948,17.0912199219507,-15.0907593677015));
#47072=CARTESIAN_POINT('Ctrl Pts',(20.0983923000268,17.0448897415811,-15.0950755304404));
#47073=CARTESIAN_POINT('Ctrl Pts',(20.0272344785269,17.000068761964,-15.0992510946321));
#47074=CARTESIAN_POINT('Ctrl Pts',(19.9539170439586,16.9587900948023,-15.1034266588238));
#47075=CARTESIAN_POINT('Ctrl Pts',(19.8788322516137,16.921249114933,-15.1076022230155));
#47076=CARTESIAN_POINT('Ctrl Pts',(19.7999551049048,16.8818120294157,-15.111988685028));
#47077=CARTESIAN_POINT('Ctrl Pts',(19.7191279049099,16.846500369128,-15.1163751470405));
#47078=CARTESIAN_POINT('Ctrl Pts',(19.6368272386529,16.8154827328641,-15.1207616090531));
#47079=CARTESIAN_POINT('Ctrl Pts',(19.5545265723959,16.7844650966001,-15.1251480710656));
#47080=CARTESIAN_POINT('Ctrl Pts',(19.470753015767,16.7577415882257,-15.1295345330781));
#47081=CARTESIAN_POINT('Ctrl Pts',(19.3859971465604,16.7354193164275,-15.1339209950907));
#47082=CARTESIAN_POINT('Ctrl Pts',(19.3051410205342,16.7141241254443,-15.1381056294837));
#47083=CARTESIAN_POINT('Ctrl Pts',(19.2230900288855,16.6967547916185,-15.1422902638768));
#47084=CARTESIAN_POINT('Ctrl Pts',(19.140260221412,16.6834413691275,-15.1464748982698));
#47085=CARTESIAN_POINT('Ctrl Pts',(19.0575483119171,16.6701468966454,-15.1506535763538));
#47086=CARTESIAN_POINT('Ctrl Pts',(18.9740602388407,16.66089694071,-15.1548322544377));
#47087=CARTESIAN_POINT('Ctrl Pts',(18.8902255245013,16.6557713242267,-15.1590109325216));
#47088=CARTESIAN_POINT('Ctrl Pts',(18.8048881331583,16.6505538347516,-15.1632645104071));
#47089=CARTESIAN_POINT('Ctrl Pts',(18.7191920174707,16.6496101194126,-15.1675180882925));
#47090=CARTESIAN_POINT('Ctrl Pts',(18.6335993142648,16.652969565798,-15.171771666178));
#47091=CARTESIAN_POINT('Ctrl Pts',(18.549665992631,16.6562638827597,-15.1759427801559));
#47092=CARTESIAN_POINT('Ctrl Pts',(18.4658325904041,16.6636959811426,-15.1801138941339));
#47093=CARTESIAN_POINT('Ctrl Pts',(18.3825365202428,16.6752410559367,-15.1842850081118));
#47094=CARTESIAN_POINT('Ctrl Pts',(18.2992684008824,16.6867822566694,-15.1884547224322));
#47095=CARTESIAN_POINT('Ctrl Pts',(18.2165377107927,16.70243362971,-15.1926244367525));
#47096=CARTESIAN_POINT('Ctrl Pts',(18.1347761196918,16.7221185762941,-15.1967941510729));
#47097=CARTESIAN_POINT('Ctrl Pts',(18.0530174380192,16.7418028224032,-15.200963717017));
#47098=CARTESIAN_POINT('Ctrl Pts',(17.9722282338244,16.7655202481684,-15.205133282961));
#47099=CARTESIAN_POINT('Ctrl Pts',(17.8928280294743,16.7931435700187,-15.209302848905));
#47100=CARTESIAN_POINT('Ctrl Pts',(17.8106362118899,16.8217380937883,-15.213619011644));
#47101=CARTESIAN_POINT('Ctrl Pts',(17.7299333840843,16.8545181133117,-15.2179351743829));
#47102=CARTESIAN_POINT('Ctrl Pts',(17.6511637413086,16.891287596088,-15.2222513371218));
#47103=CARTESIAN_POINT('Ctrl Pts',(17.5749600113613,16.9268593168303,-15.2264269013135));
#47104=CARTESIAN_POINT('Ctrl Pts',(17.5005658480124,16.966164316944,-15.2306024655052));
#47105=CARTESIAN_POINT('Ctrl Pts',(17.4283578509306,17.0089785244977,-15.2347780296969));
#47106=CARTESIAN_POINT('Ctrl Pts',(17.3525027995743,17.0539551758939,-15.2391644917094));
#47107=CARTESIAN_POINT('Ctrl Pts',(17.2790610511154,17.1028045279329,-15.243550953722));
#47108=CARTESIAN_POINT('Ctrl Pts',(17.2084323379752,17.1552171056787,-15.2479374157345));
#47109=CARTESIAN_POINT('Ctrl Pts',(17.137803624835,17.2076296834245,-15.252323877747));
#47110=CARTESIAN_POINT('Ctrl Pts',(17.0699883460668,17.2636050588652,-15.2567103397596));
#47111=CARTESIAN_POINT('Ctrl Pts',(17.0053421035811,17.3227887096121,-15.2610968017721));
#47112=CARTESIAN_POINT('Ctrl Pts',(16.9445899812052,17.3784072924496,-15.2652190348167));
#47113=CARTESIAN_POINT('Ctrl Pts',(16.8863955977243,17.4370795204071,-15.2693412678613));
#47114=CARTESIAN_POINT('Ctrl Pts',(16.8310887538612,17.4985372152019,-15.2734635009059));
#47115=CARTESIAN_POINT('Ctrl Pts',(16.7758743514516,17.5598921878336,-15.2775788439313));
#47116=CARTESIAN_POINT('Ctrl Pts',(16.7235382140142,17.6240230272318,-15.2816941869568));
#47117=CARTESIAN_POINT('Ctrl Pts',(16.6743754759291,17.6906228034315,-15.2858095299822));
#47118=CARTESIAN_POINT('Ctrl Pts',(16.6252589923635,17.7571599195604,-15.2899210011074));
#47119=CARTESIAN_POINT('Ctrl Pts',(16.5793102664133,17.8261609852053,-15.2940324722327));
#47120=CARTESIAN_POINT('Ctrl Pts',(16.5367853878605,17.8972846776411,-15.2981439433579));
#47121=CARTESIAN_POINT('Ctrl Pts',(16.4942868717928,17.9683642783041,-15.3022528656553));
#47122=CARTESIAN_POINT('Ctrl Pts',(16.4552082342176,18.0415634879277,-15.3063617879526));
#47123=CARTESIAN_POINT('Ctrl Pts',(16.4197623875935,18.1165118669794,-15.31047071025));
#47124=CARTESIAN_POINT('Ctrl Pts',(16.3843271437776,18.1914378269504,-15.3145784034579));
#47125=CARTESIAN_POINT('Ctrl Pts',(16.3525227351488,18.2681114878987,-15.3186860966658));
#47126=CARTESIAN_POINT('Ctrl Pts',(16.3245154961046,18.3461390715913,-15.3227937898737));
#47127=CARTESIAN_POINT('Ctrl Pts',(16.2964946934756,18.4242044431483,-15.3269034723904));
#47128=CARTESIAN_POINT('Ctrl Pts',(16.2722748983311,18.5036246009546,-15.331013154907));
#47129=CARTESIAN_POINT('Ctrl Pts',(16.2519734104525,18.5839880313907,-15.3351228374237));
#47130=CARTESIAN_POINT('Ctrl Pts',(16.2316667383952,18.664371983396,-15.339233569387));
#47131=CARTESIAN_POINT('Ctrl Pts',(16.2152804642371,18.7456992225571,-15.3433443013503));
#47132=CARTESIAN_POINT('Ctrl Pts',(16.2028808242116,18.8275476327413,-15.3474550333136));
#47133=CARTESIAN_POINT('Ctrl Pts',(16.1904661338127,18.9094953884816,-15.3515707547807));
#47134=CARTESIAN_POINT('Ctrl Pts',(16.1820477886727,18.9919651056506,-15.3556864762478));
#47135=CARTESIAN_POINT('Ctrl Pts',(16.1776401048969,19.0745299054429,-15.3598021977149));
#47136=CARTESIAN_POINT('Ctrl Pts',(16.175174200724,19.1207212600628,-15.3621047618861));
#47137=CARTESIAN_POINT('Ctrl Pts',(16.173962657598,19.1669423575626,-15.3644073260573));
#47138=CARTESIAN_POINT('Ctrl Pts',(16.1740008768645,19.213118854712,-15.3667098902285));
#47139=CARTESIAN_POINT('Origin',(18.734,19.211,1.76670989022852));
#47140=CARTESIAN_POINT('',(20.2909850521016,21.2378231040073,-14.0501277863708));
#47141=CARTESIAN_POINT('',(20.2961055941918,21.2444717899281,-14.1167030457843));
#47142=CARTESIAN_POINT('',(20.2935358855687,21.2411349269503,1.76670989022852));
#47143=CARTESIAN_POINT('',(16.1738766799073,19.2098698167329,-14.6332901097715));
#47144=CARTESIAN_POINT('Ctrl Pts',(20.2961055941918,21.2444717899281,-14.1167030457843));
#47145=CARTESIAN_POINT('Ctrl Pts',(20.9598513200281,20.733315419597,-14.1585606280004));
#47146=CARTESIAN_POINT('Ctrl Pts',(21.7469835110905,18.9872885505905,-14.2428101457769));
#47147=CARTESIAN_POINT('Ctrl Pts',(20.188947426677,16.556490896078,-14.369451599114));
#47148=CARTESIAN_POINT('Ctrl Pts',(17.2895133755746,16.5507840333809,-14.4966274057954));
#47149=CARTESIAN_POINT('Ctrl Pts',(16.200898327955,18.2345794040693,-14.5845735760146));
#47150=CARTESIAN_POINT('Ctrl Pts',(16.1700292343928,19.1465375881033,-14.6301278106733));
#47151=CARTESIAN_POINT('Ctrl Pts',(16.1703790132248,19.209868272665,-14.6332901097715));
#47152=CARTESIAN_POINT('Ctrl Pts',(16.1740002494514,19.2098698712835,-14.6332901097715));
#47153=CARTESIAN_POINT('Ctrl Pts',(16.1739637014967,19.2926593390013,-14.6374299052976));
#47154=CARTESIAN_POINT('Ctrl Pts',(16.1779474618949,19.3756125071059,-14.6415697008237));
#47155=CARTESIAN_POINT('Ctrl Pts',(16.1859729132155,19.4583013647604,-14.6457094963498));
#47156=CARTESIAN_POINT('Ctrl Pts',(16.1939875490477,19.5408787868903,-14.6498437128862));
#47157=CARTESIAN_POINT('Ctrl Pts',(16.2060330170348,19.6231921412973,-14.6539779294227));
#47158=CARTESIAN_POINT('Ctrl Pts',(16.2220786798975,19.7048130026784,-14.6581121459591));
#47159=CARTESIAN_POINT('Ctrl Pts',(16.2381078732804,19.7863500873324,-14.6622421190812));
#47160=CARTESIAN_POINT('Ctrl Pts',(16.2581290152452,19.8671956313601,-14.6663720922033));
#47161=CARTESIAN_POINT('Ctrl Pts',(16.2820597821147,19.9469274202778,-14.6705020653254));
#47162=CARTESIAN_POINT('Ctrl Pts',(16.3059775967094,20.0266160552067,-14.6746298031431));
#47163=CARTESIAN_POINT('Ctrl Pts',(16.3338007023326,20.1051916814476,-14.6787575409609));
#47164=CARTESIAN_POINT('Ctrl Pts',(16.3653962152437,20.1822446194642,-14.6828852787787));
#47165=CARTESIAN_POINT('Ctrl Pts',(16.3969845852851,20.2592801379472,-14.6870120834293));
#47166=CARTESIAN_POINT('Ctrl Pts',(16.4323434905921,20.3347932165774,-14.69113888808));
#47167=CARTESIAN_POINT('Ctrl Pts',(16.4712914723381,20.4083930511099,-14.6952656927307));
#47168=CARTESIAN_POINT('Ctrl Pts',(16.5102429241535,20.4819994430175,-14.6993928650588));
#47169=CARTESIAN_POINT('Ctrl Pts',(16.5527838651363,20.5536918375771,-14.703520037387));
#47170=CARTESIAN_POINT('Ctrl Pts',(16.5986870593961,20.6231043324377,-14.7076472097152));
#47171=CARTESIAN_POINT('Ctrl Pts',(16.6446377721104,20.6925886823084,-14.7117786544444));
#47172=CARTESIAN_POINT('Ctrl Pts',(16.6939574240325,20.7597880294055,-14.7159100991735));
#47173=CARTESIAN_POINT('Ctrl Pts',(16.7463760416131,20.8243663564257,-14.7200415439027));
#47174=CARTESIAN_POINT('Ctrl Pts',(16.7988250781885,20.8889821588294,-14.7241753861463));
#47175=CARTESIAN_POINT('Ctrl Pts',(16.8543763437708,20.9509735655353,-14.7283092283899));
#47176=CARTESIAN_POINT('Ctrl Pts',(16.9127219511763,21.0100403744422,-14.7324430706336));
#47177=CARTESIAN_POINT('Ctrl Pts',(16.9711635405887,21.0692043517755,-14.7365837132945));
#47178=CARTESIAN_POINT('Ctrl Pts',(17.0324082986529,21.1254338132414,-14.7407243559553));
#47179=CARTESIAN_POINT('Ctrl Pts',(17.0961145829399,21.1784682616454,-14.7448649986162));
#47180=CARTESIAN_POINT('Ctrl Pts',(17.1274705472745,21.2045715933853,-14.7469030054636));
#47181=CARTESIAN_POINT('Ctrl Pts',(17.1594223751536,21.2299015689542,-14.7489410123109));
#47182=CARTESIAN_POINT('Ctrl Pts',(17.1919269101815,21.2544310817,-14.7509790191583));
#47183=CARTESIAN_POINT('Ctrl Pts',(17.2586683911457,21.3047974692387,-14.7551636535514));
#47184=CARTESIAN_POINT('Ctrl Pts',(17.3280042311,21.3519843348469,-14.7593482879444));
#47185=CARTESIAN_POINT('Ctrl Pts',(17.3995987737075,21.395713566413,-14.7635329223375));
#47186=CARTESIAN_POINT('Ctrl Pts',(17.4710914103449,21.4393805548304,-14.7677116004214));
#47187=CARTESIAN_POINT('Ctrl Pts',(17.5448359744303,21.4795994471399,-14.7718902785053));
#47188=CARTESIAN_POINT('Ctrl Pts',(17.6204652949927,21.5161335017183,-14.7760689565893));
#47189=CARTESIAN_POINT('Ctrl Pts',(17.6974502167725,21.5533224029686,-14.7803225344747));
#47190=CARTESIAN_POINT('Ctrl Pts',(17.7763877432988,21.5866927752842,-14.7845761123601));
#47191=CARTESIAN_POINT('Ctrl Pts',(17.8568613993343,21.616042177431,-14.7888296902455));
#47192=CARTESIAN_POINT('Ctrl Pts',(17.9357749165162,21.6448225841466,-14.7930008042235));
#47193=CARTESIAN_POINT('Ctrl Pts',(18.0161650808992,21.6697363732161,-14.7971719182015));
#47194=CARTESIAN_POINT('Ctrl Pts',(18.0976177441658,21.6906406240541,-14.8013430321794));
#47195=CARTESIAN_POINT('Ctrl Pts',(18.1790430752045,21.7115378602688,-14.8055127464998));
#47196=CARTESIAN_POINT('Ctrl Pts',(18.2615297518276,21.7284281160528,-14.8096824608201));
#47197=CARTESIAN_POINT('Ctrl Pts',(18.34464929881,21.7412185738554,-14.8138521751405));
#47198=CARTESIAN_POINT('Ctrl Pts',(18.4277658880424,21.7540085765186,-14.8180217410846));
#47199=CARTESIAN_POINT('Ctrl Pts',(18.5115148480473,21.7626990021398,-14.8221913070286));
#47200=CARTESIAN_POINT('Ctrl Pts',(18.5954597232797,21.7672485387235,-14.8263608729727));
#47201=CARTESIAN_POINT('Ctrl Pts',(18.6823559967678,21.7719580314011,-14.8306770357116));
#47202=CARTESIAN_POINT('Ctrl Pts',(18.7694616919208,21.7722300013651,-14.8349931984505));
#47203=CARTESIAN_POINT('Ctrl Pts',(18.8562914526108,21.7680773943349,-14.8393093611894));
#47204=CARTESIAN_POINT('Ctrl Pts',(18.9402927429791,21.7640600580418,-14.8434849253811));
#47205=CARTESIAN_POINT('Ctrl Pts',(19.0240353356991,21.7559020718403,-14.8476604895728));
#47206=CARTESIAN_POINT('Ctrl Pts',(19.1070857885135,21.7436679597628,-14.8518360537644));
#47207=CARTESIAN_POINT('Ctrl Pts',(19.1943309222659,21.7308159317682,-14.856222515777));
#47208=CARTESIAN_POINT('Ctrl Pts',(19.2808115861344,21.7134653009972,-14.8606089777895));
#47209=CARTESIAN_POINT('Ctrl Pts',(19.3660405469233,21.691750843403,-14.864995439802));
#47210=CARTESIAN_POINT('Ctrl Pts',(19.4512695077122,21.6700363858089,-14.8693819018146));
#47211=CARTESIAN_POINT('Ctrl Pts',(19.5352462338658,21.6439583461085,-14.8737683638271));
#47212=CARTESIAN_POINT('Ctrl Pts',(19.6175072439392,21.6137099179691,-14.8781548258396));
#47213=CARTESIAN_POINT('Ctrl Pts',(19.6959730538369,21.5848570335956,-14.8823389137094));
#47214=CARTESIAN_POINT('Ctrl Pts',(19.7731699980662,21.5521027093326,-14.8865230015791));
#47215=CARTESIAN_POINT('Ctrl Pts',(19.8486827058602,21.5155785873466,-14.8907070894488));
#47216=CARTESIAN_POINT('Ctrl Pts',(19.9270438215451,21.4776767423214,-14.8950490049114));
#47217=CARTESIAN_POINT('Ctrl Pts',(20.003590624008,21.4357151321965,-14.899390920374));
#47218=CARTESIAN_POINT('Ctrl Pts',(20.0778772783341,21.3898973956516,-14.9037328358367));
#47219=CARTESIAN_POINT('Ctrl Pts',(20.1521639326601,21.3440796591068,-14.9080747512993));
#47220=CARTESIAN_POINT('Ctrl Pts',(20.2241899272934,21.2944060218976,-14.9124166667619));
#47221=CARTESIAN_POINT('Ctrl Pts',(20.2935358855687,21.2411349269503,-14.9167585822245));
#47222=CARTESIAN_POINT('',(16.17436451349,19.211560173865,-14.5667099150528));
#47223=CARTESIAN_POINT('Ctrl Pts',(16.1740000613162,19.211560302475,-14.5667099174729));
#47224=CARTESIAN_POINT('Ctrl Pts',(16.1740197372987,19.30145909156,-14.5711571992719));
#47225=CARTESIAN_POINT('Ctrl Pts',(16.1787790795977,19.3912344818004,-14.5756044810709));
#47226=CARTESIAN_POINT('Ctrl Pts',(16.1882138900509,19.4803939167657,-14.5800517628699));
#47227=CARTESIAN_POINT('Ctrl Pts',(16.1976832329532,19.5698796851174,-14.5845153222118));
#47228=CARTESIAN_POINT('Ctrl Pts',(16.2118622325346,19.6587446305158,-14.5889788815537));
#47229=CARTESIAN_POINT('Ctrl Pts',(16.2306352202496,19.7465042292131,-14.5934424408955));
#47230=CARTESIAN_POINT('Ctrl Pts',(16.2494446598929,19.8344342326776,-14.59791466723));
#47231=CARTESIAN_POINT('Ctrl Pts',(16.2728657964751,19.9212542602436,-14.6023868935645));
#47232=CARTESIAN_POINT('Ctrl Pts',(16.3007333122769,20.0064955854165,-14.606859119899));
#47233=CARTESIAN_POINT('Ctrl Pts',(16.3286838403156,20.0919908289195,-14.6113446681784));
#47234=CARTESIAN_POINT('Ctrl Pts',(16.3611071025133,20.175897631469,-14.6158302164578));
#47235=CARTESIAN_POINT('Ctrl Pts',(16.3977895032108,20.2577666954446,-14.6203157647373));
#47236=CARTESIAN_POINT('Ctrl Pts',(16.4111522146037,20.2875900617759,-14.6219497659465));
#47237=CARTESIAN_POINT('Ctrl Pts',(16.4250796827617,20.3171432681483,-14.6235837671557));
#47238=CARTESIAN_POINT('Ctrl Pts',(16.4395601204677,20.3464054955,-14.625217768365));
#47239=CARTESIAN_POINT('Ctrl Pts',(16.4766441429939,20.4213452949944,-14.629402402758));
#47240=CARTESIAN_POINT('Ctrl Pts',(16.5174725051856,20.4946058152549,-14.633587037151));
#47241=CARTESIAN_POINT('Ctrl Pts',(16.5618698248528,20.5657879916116,-14.6377716715441));
#47242=CARTESIAN_POINT('Ctrl Pts',(16.6062039504308,20.636868848951,-14.641950349628));
#47243=CARTESIAN_POINT('Ctrl Pts',(16.6540967016935,20.7058768514384,-14.646129027712));
#47244=CARTESIAN_POINT('Ctrl Pts',(16.7053259809371,20.7724357893872,-14.6503077057959));
#47245=CARTESIAN_POINT('Ctrl Pts',(16.7574735081934,20.8401877484638,-14.6545612836814));
#47246=CARTESIAN_POINT('Ctrl Pts',(16.8130781406444,20.9054015483267,-14.6588148615668));
#47247=CARTESIAN_POINT('Ctrl Pts',(16.8718583319471,20.9677095400496,-14.6630684394523));
#47248=CARTESIAN_POINT('Ctrl Pts',(16.9294989545412,21.0288095697688,-14.6672395534302));
#47249=CARTESIAN_POINT('Ctrl Pts',(16.9901927757377,21.0871151053885,-14.6714106674082));
#47250=CARTESIAN_POINT('Ctrl Pts',(17.0536336491124,21.1423127470207,-14.6755817813861));
#47251=CARTESIAN_POINT('Ctrl Pts',(17.1170532342894,21.1974918665512,-14.6797514957065));
#47252=CARTESIAN_POINT('Ctrl Pts',(17.1832176941668,21.249564861567,-14.6839212100268));
#47253=CARTESIAN_POINT('Ctrl Pts',(17.2517856166925,21.2982566976576,-14.6880909243472));
#47254=CARTESIAN_POINT('Ctrl Pts',(17.3203510992774,21.3469468010837,-14.6922604902913));
#47255=CARTESIAN_POINT('Ctrl Pts',(17.3913194988898,21.3922557191442,-14.6964300562353));
#47256=CARTESIAN_POINT('Ctrl Pts',(17.4643191824367,21.4339508814888,-14.7005996221793));
#47257=CARTESIAN_POINT('Ctrl Pts',(17.5398854448023,21.4771119943049,-14.7049157849183));
#47258=CARTESIAN_POINT('Ctrl Pts',(17.6176280306767,21.5164002423865,-14.7092319476572));
#47259=CARTESIAN_POINT('Ctrl Pts',(17.6971072733111,21.5516096371116,-14.7135481103961));
#47260=CARTESIAN_POINT('Ctrl Pts',(17.7739974879763,21.5856720895068,-14.7177236745878));
#47261=CARTESIAN_POINT('Ctrl Pts',(17.8525124972024,21.6159172197027,-14.7218992387795));
#47262=CARTESIAN_POINT('Ctrl Pts',(17.9322359204944,21.6422084157502,-14.7260748029711));
#47263=CARTESIAN_POINT('Ctrl Pts',(18.0159859843726,21.6698275176087,-14.7304612649837));
#47264=CARTESIAN_POINT('Ctrl Pts',(18.1010691812453,21.6930826078308,-14.7348477269962));
#47265=CARTESIAN_POINT('Ctrl Pts',(18.1869895560291,21.7118757614457,-14.7392341890088));
#47266=CARTESIAN_POINT('Ctrl Pts',(18.2729099308129,21.7306689150606,-14.7436206510213));
#47267=CARTESIAN_POINT('Ctrl Pts',(18.3596668986516,21.7450001125529,-14.7480071130339));
#47268=CARTESIAN_POINT('Ctrl Pts',(18.4467595506039,21.7548342957494,-14.7523935750464));
#47269=CARTESIAN_POINT('Ctrl Pts',(18.5298216106109,21.7642133592694,-14.7565770344168));
#47270=CARTESIAN_POINT('Ctrl Pts',(18.6134980569014,21.7695373443218,-14.7607604937872));
#47271=CARTESIAN_POINT('Ctrl Pts',(18.6973587722112,21.7707377639958,-14.7649439531576));
#47272=CARTESIAN_POINT('Ctrl Pts',(18.7811102468207,21.7719366199497,-14.7691219629677));
#47273=CARTESIAN_POINT('Ctrl Pts',(18.8650450584586,21.7690225671106,-14.7732999727777));
#47274=CARTESIAN_POINT('Ctrl Pts',(18.9487268680233,21.761978708682,-14.7774779825878));
#47275=CARTESIAN_POINT('Ctrl Pts',(19.0323247810394,21.7549419121873,-14.7816518036666));
#47276=CARTESIAN_POINT('Ctrl Pts',(19.1156697399229,21.743783570225,-14.7858256247455));
#47277=CARTESIAN_POINT('Ctrl Pts',(19.1983256615625,21.7285388140036,-14.7899994458244));
#47278=CARTESIAN_POINT('Ctrl Pts',(19.2809235142162,21.7133047678138,-14.7941703346324));
#47279=CARTESIAN_POINT('Ctrl Pts',(19.3628328402605,21.693990093863,-14.7983412234403));
#47280=CARTESIAN_POINT('Ctrl Pts',(19.4436242958245,21.6706815563759,-14.8025121122483));
#47281=CARTESIAN_POINT('Ctrl Pts',(19.5244040000542,21.6473764091781,-14.8066823943892));
#47282=CARTESIAN_POINT('Ctrl Pts',(19.6040657115569,21.6200786673617,-14.8108526765302));
#47283=CARTESIAN_POINT('Ctrl Pts',(19.6821928869638,21.588925618919,-14.8150229586712));
#47284=CARTESIAN_POINT('Ctrl Pts',(19.7603101594136,21.5577765192598,-14.8191927122108));
#47285=CARTESIAN_POINT('Ctrl Pts',(19.8368928571116,21.5227732602624,-14.8233624657505));
#47286=CARTESIAN_POINT('Ctrl Pts',(19.9115437773165,21.4841015490961,-14.8275322192902));
#47287=CARTESIAN_POINT('Ctrl Pts',(19.9862468140608,21.445402839793,-14.8317048838875));
#47288=CARTESIAN_POINT('Ctrl Pts',(20.0590149720293,21.4030307779422,-14.8358775484847));
#47289=CARTESIAN_POINT('Ctrl Pts',(20.129475672665,21.3572170549597,-14.8400502130819));
#47290=CARTESIAN_POINT('Ctrl Pts',(20.1856889996356,21.3206670098067,-14.8433791518695));
#47291=CARTESIAN_POINT('Ctrl Pts',(20.2404341027343,21.2819273564674,-14.846708090657));
#47292=CARTESIAN_POINT('Ctrl Pts',(20.2935358855687,21.2411349269503,-14.8500370294445));
#47293=CARTESIAN_POINT('Ctrl Pts',(20.2909850521016,21.2378231040073,-14.0501277863708));
#47294=CARTESIAN_POINT('Ctrl Pts',(20.6448529615788,20.9653099953601,-14.0722567047936));
#47295=CARTESIAN_POINT('Ctrl Pts',(21.48038594828,19.9142910878859,-14.1367775587769));
#47296=CARTESIAN_POINT('Ctrl Pts',(21.2244734734613,17.4902926282723,-14.2436903483206));
#47297=CARTESIAN_POINT('Ctrl Pts',(18.6352034638416,16.1855196702712,-14.3708661550021));
#47298=CARTESIAN_POINT('Ctrl Pts',(16.5197423492181,17.430869440195,-14.478539335638));
#47299=CARTESIAN_POINT('Ctrl Pts',(16.1790023518676,18.7496082788979,-14.5438205807135));
#47300=CARTESIAN_POINT('Ctrl Pts',(16.1781028428963,19.2115588546613,-14.5667098902285));
#47301=CARTESIAN_POINT('Origin',(18.734,19.211,1.76670989022852));
#47302=CARTESIAN_POINT('',(20.2935358855687,21.2411349269503,-13.2501880127039));
#47303=CARTESIAN_POINT('',(20.2935358855687,21.2411349269503,-13.3166223773735));
#47304=CARTESIAN_POINT('',(20.2935358855687,21.2411349269503,1.76670989022852));
#47305=CARTESIAN_POINT('',(16.1740010575059,19.2133268925441,-13.8332901097715));
#47306=CARTESIAN_POINT('Ctrl Pts',(20.2935358855687,21.2411349269503,-13.3166223773735));
#47307=CARTESIAN_POINT('Ctrl Pts',(20.3602103291409,21.1899160714837,-13.3207986505334));
#47308=CARTESIAN_POINT('Ctrl Pts',(20.4243042199467,21.1354511939907,-13.3249749236932));
#47309=CARTESIAN_POINT('Ctrl Pts',(20.4855003216615,21.07804221249,-13.329151196853));
#47310=CARTESIAN_POINT('Ctrl Pts',(20.5468041075984,21.0205322108043,-13.3333348188261));
#47311=CARTESIAN_POINT('Ctrl Pts',(20.6051995980666,20.9600680873566,-13.3375184407992));
#47312=CARTESIAN_POINT('Ctrl Pts',(20.6604076888247,20.8969873713753,-13.3417020627724));
#47313=CARTESIAN_POINT('Ctrl Pts',(20.7059042993841,20.8450029841342,-13.3451497570691));
#47314=CARTESIAN_POINT('Ctrl Pts',(20.7492369226164,20.7912423162171,-13.3485974513658));
#47315=CARTESIAN_POINT('Ctrl Pts',(20.7902715950829,20.7359088914605,-13.3520451456625));
#47316=CARTESIAN_POINT('Ctrl Pts',(20.8400773745207,20.6687480203407,-13.3562297800555));
#47317=CARTESIAN_POINT('Ctrl Pts',(20.886682020299,20.5990195040797,-13.3604144144486));
#47318=CARTESIAN_POINT('Ctrl Pts',(20.9298102405871,20.5270613159473,-13.3645990488416));
#47319=CARTESIAN_POINT('Ctrl Pts',(20.9728770731918,20.4552055513889,-13.3687777269256));
#47320=CARTESIAN_POINT('Ctrl Pts',(21.0124770746365,20.3811268100632,-13.3729564050095));
#47321=CARTESIAN_POINT('Ctrl Pts',(21.0483765860078,20.3051942323642,-13.3771350830935));
#47322=CARTESIAN_POINT('Ctrl Pts',(21.0849195703198,20.2279006177817,-13.3813886609789));
#47323=CARTESIAN_POINT('Ctrl Pts',(21.1176278099319,20.1486864403634,-13.3856422388643));
#47324=CARTESIAN_POINT('Ctrl Pts',(21.1463023579537,20.0679698558355,-13.3898958167498));
#47325=CARTESIAN_POINT('Ctrl Pts',(21.1744209939084,19.9888181198042,-13.3940669307277));
#47326=CARTESIAN_POINT('Ctrl Pts',(21.1986607834443,19.9082221644554,-13.3982380447057));
#47327=CARTESIAN_POINT('Ctrl Pts',(21.2188822787495,19.8265973202967,-13.4024091586836));
#47328=CARTESIAN_POINT('Ctrl Pts',(21.2390969885367,19.7449998661427,-13.406578873004));
#47329=CARTESIAN_POINT('Ctrl Pts',(21.2552959714612,19.6623746550204,-13.4107485873244));
#47330=CARTESIAN_POINT('Ctrl Pts',(21.2673900009521,19.5791509243178,-13.4149183016447));
#47331=CARTESIAN_POINT('Ctrl Pts',(21.2794836000854,19.4959301550728,-13.4190878675888));
#47332=CARTESIAN_POINT('Ctrl Pts',(21.2874724709,19.4121113639668,-13.4232574335328));
#47333=CARTESIAN_POINT('Ctrl Pts',(21.2913189573957,19.3281313371597,-13.4274269994769));
#47334=CARTESIAN_POINT('Ctrl Pts',(21.2953006816113,19.2411986762106,-13.4317431622158));
#47335=CARTESIAN_POINT('Ctrl Pts',(21.2948432851383,19.1540937573815,-13.4360593249547));
#47336=CARTESIAN_POINT('Ctrl Pts',(21.2899637772452,19.0673018113879,-13.4403754876936));
#47337=CARTESIAN_POINT('Ctrl Pts',(21.2852432188086,18.9833371039062,-13.4445510518853));
#47338=CARTESIAN_POINT('Ctrl Pts',(21.2763843217563,18.89966575566,-13.448726616077));
#47339=CARTESIAN_POINT('Ctrl Pts',(21.2634552371753,18.8167206534363,-13.4529021802687));
#47340=CARTESIAN_POINT('Ctrl Pts',(21.249873135268,18.7295861912824,-13.4572886422812));
#47341=CARTESIAN_POINT('Ctrl Pts',(21.2317989893781,18.6432538400943,-13.4616751042937));
#47342=CARTESIAN_POINT('Ctrl Pts',(21.2093716504547,18.5582096874759,-13.4660615663063));
#47343=CARTESIAN_POINT('Ctrl Pts',(21.1869443115313,18.4731655348574,-13.4704480283188));
#47344=CARTESIAN_POINT('Ctrl Pts',(21.1601640287335,18.3894101102965,-13.4748344903314));
#47345=CARTESIAN_POINT('Ctrl Pts',(21.1292278697973,18.3074052613331,-13.4792209523439));
#47346=CARTESIAN_POINT('Ctrl Pts',(21.0997151293921,18.2291735770309,-13.4834055867369));
#47347=CARTESIAN_POINT('Ctrl Pts',(21.0663106928263,18.1522437219301,-13.48759022113));
#47348=CARTESIAN_POINT('Ctrl Pts',(21.0291497318876,18.0770301114155,-13.491774855523));
#47349=CARTESIAN_POINT('Ctrl Pts',(20.9920416649771,18.0019235581658,-13.495953533607));
#47350=CARTESIAN_POINT('Ctrl Pts',(20.9511878964457,17.9285288061218,-13.5001322116909));
#47351=CARTESIAN_POINT('Ctrl Pts',(20.9067723398089,17.8572421341461,-13.5043108897749));
#47352=CARTESIAN_POINT('Ctrl Pts',(20.8615606662404,17.7846776998082,-13.5085644676603));
#47353=CARTESIAN_POINT('Ctrl Pts',(20.8126584286881,17.7142981146648,-13.5128180455458));
#47354=CARTESIAN_POINT('Ctrl Pts',(20.7603095437651,17.6464970013302,-13.5170716234312));
#47355=CARTESIAN_POINT('Ctrl Pts',(20.7089755441266,17.5800103448805,-13.5212427374092));
#47356=CARTESIAN_POINT('Ctrl Pts',(20.6543276385964,17.5160034559035,-13.5254138513871));
#47357=CARTESIAN_POINT('Ctrl Pts',(20.5966395739482,17.4548183984673,-13.5295849653651));
#47358=CARTESIAN_POINT('Ctrl Pts',(20.5389708670873,17.3936538722681,-13.5337546796854));
#47359=CARTESIAN_POINT('Ctrl Pts',(20.4782643424756,17.3353096315038,-13.5379243940058));
#47360=CARTESIAN_POINT('Ctrl Pts',(20.4148326241777,17.2800930396573,-13.5420941083262));
#47361=CARTESIAN_POINT('Ctrl Pts',(20.3514031630525,17.224878412654,-13.5462636742702));
#47362=CARTESIAN_POINT('Ctrl Pts',(20.2852490485945,17.1727915146886,-13.5504332402143));
#47363=CARTESIAN_POINT('Ctrl Pts',(20.2167171663627,17.1241004325619,-13.5546028061583));
#47364=CARTESIAN_POINT('Ctrl Pts',(20.145775787695,17.0736974320547,-13.5589189688972));
#47365=CARTESIAN_POINT('Ctrl Pts',(20.0722867555764,17.0269337896173,-13.5632351316361));
#47366=CARTESIAN_POINT('Ctrl Pts',(19.9966672790437,16.9840578493296,-13.5675512943751));
#47367=CARTESIAN_POINT('Ctrl Pts',(19.9235110990054,16.9425785882871,-13.5717268585667));
#47368=CARTESIAN_POINT('Ctrl Pts',(19.8483615834561,16.9047378049042,-13.5759024227584));
#47369=CARTESIAN_POINT('Ctrl Pts',(19.7716196105687,16.8707125083094,-13.5800779869501));
#47370=CARTESIAN_POINT('Ctrl Pts',(19.6910015830675,16.8349686748712,-13.5844644489626));
#47371=CARTESIAN_POINT('Ctrl Pts',(19.6086265457422,16.8034361069935,-13.5888509109752));
#47372=CARTESIAN_POINT('Ctrl Pts',(19.524978378728,16.7762611630023,-13.5932373729877));
#47373=CARTESIAN_POINT('Ctrl Pts',(19.4413302117138,16.7490862190112,-13.5976238350002));
#47374=CARTESIAN_POINT('Ctrl Pts',(19.3564094950912,16.7262689760049,-13.6020102970128));
#47375=CARTESIAN_POINT('Ctrl Pts',(19.2707112385803,16.7078937205181,-13.6063967590253));
#47376=CARTESIAN_POINT('Ctrl Pts',(19.1889560858867,16.6903639377749,-13.6105813934184));
#47377=CARTESIAN_POINT('Ctrl Pts',(19.1061890642126,16.676811111084,-13.6147660278114));
#47378=CARTESIAN_POINT('Ctrl Pts',(19.0228317972389,16.6673458975514,-13.6189506622045));
#47379=CARTESIAN_POINT('Ctrl Pts',(18.9395931790174,16.6578941565786,-13.6231293402884));
#47380=CARTESIAN_POINT('Ctrl Pts',(18.8557664374668,16.6525185234246,-13.6273080183724));
#47381=CARTESIAN_POINT('Ctrl Pts',(18.771784329296,16.6512788541602,-13.6314866964563));
#47382=CARTESIAN_POINT('Ctrl Pts',(18.6862969021931,16.6500169647151,-13.6357402743417));
#47383=CARTESIAN_POINT('Ctrl Pts',(18.6006489552155,16.6530408729659,-13.6399938522272));
#47384=CARTESIAN_POINT('Ctrl Pts',(18.5153034901262,16.6603585440974,-13.6442474301126));
#47385=CARTESIAN_POINT('Ctrl Pts',(18.4316126134156,16.6675343478947,-13.6484185440906));
#47386=CARTESIAN_POINT('Ctrl Pts',(18.3482130743119,16.6788388732104,-13.6525896580685));
#47387=CARTESIAN_POINT('Ctrl Pts',(18.2655406685,16.6942270951215,-13.6567607720465));
#47388=CARTESIAN_POINT('Ctrl Pts',(18.1828960042124,16.7096101533661,-13.6609304863668));
#47389=CARTESIAN_POINT('Ctrl Pts',(18.100978440524,16.729074102609,-13.6651002006872));
#47390=CARTESIAN_POINT('Ctrl Pts',(18.0202156389592,16.7525224455095,-13.6692699150076));
#47391=CARTESIAN_POINT('Ctrl Pts',(17.9394557112815,16.7759699540173,-13.6734394809516));
#47392=CARTESIAN_POINT('Ctrl Pts',(17.8598509055789,16.8034014451982,-13.6776090468957));
#47393=CARTESIAN_POINT('Ctrl Pts',(17.7818144029991,16.8346703534938,-13.6817786128397));
#47394=CARTESIAN_POINT('Ctrl Pts',(17.701034233257,16.8670386380308,-13.6860947755786));
#47395=CARTESIAN_POINT('Ctrl Pts',(17.6219351912178,16.9035190114424,-13.6904109383175));
#47396=CARTESIAN_POINT('Ctrl Pts',(17.5449519222901,16.9438950908936,-13.6947271010565));
#47397=CARTESIAN_POINT('Ctrl Pts',(17.4704763752506,16.9829559238034,-13.6989026652481));
#47398=CARTESIAN_POINT('Ctrl Pts',(17.3979812574158,17.0256622753737,-13.7030782294398));
#47399=CARTESIAN_POINT('Ctrl Pts',(17.3278323932023,17.0717728821855,-13.7072537936315));
#47400=CARTESIAN_POINT('Ctrl Pts',(17.2541404766203,17.12021242613,-13.7116402556441));
#47401=CARTESIAN_POINT('Ctrl Pts',(17.1830385318339,17.1724088154586,-13.7160267176566));
#47402=CARTESIAN_POINT('Ctrl Pts',(17.1149115381735,17.2280344045394,-13.7204131796691));
#47403=CARTESIAN_POINT('Ctrl Pts',(17.0467845445131,17.2836599936203,-13.7247996416817));
#47404=CARTESIAN_POINT('Ctrl Pts',(16.9816328807927,17.3427143364292,-13.7291861036942));
#47405=CARTESIAN_POINT('Ctrl Pts',(16.919795358022,17.4048268308312,-13.7335725657068));
#47406=CARTESIAN_POINT('Ctrl Pts',(16.8612222805614,17.4636603639818,-13.7377274633762));
#47407=CARTESIAN_POINT('Ctrl Pts',(16.8053896617353,17.5254713783546,-13.7418823610455));
#47408=CARTESIAN_POINT('Ctrl Pts',(16.7526212754374,17.5899699725635,-13.7460372587149));
#47409=CARTESIAN_POINT('Ctrl Pts',(16.70029462084,17.6539286398257,-13.7501573751423));
#47410=CARTESIAN_POINT('Ctrl Pts',(16.650981430094,17.7205297194408,-13.7542774915697));
#47411=CARTESIAN_POINT('Ctrl Pts',(16.6049624110077,17.7894519196813,-13.7583976079971));
#47412=CARTESIAN_POINT('Ctrl Pts',(16.5589874739682,17.8583080987046,-13.7625137777266));
#47413=CARTESIAN_POINT('Ctrl Pts',(16.5163007099123,17.9294805955777,-13.7666299474561));
#47414=CARTESIAN_POINT('Ctrl Pts',(16.4771421768206,18.0026156381539,-13.7707461171856));
#47415=CARTESIAN_POINT('Ctrl Pts',(16.4380086398887,18.0757039962642,-13.7748596594307));
#47416=CARTESIAN_POINT('Ctrl Pts',(16.4023990866292,18.1507519968567,-13.7789732016757));
#47417=CARTESIAN_POINT('Ctrl Pts',(16.3705090605921,18.2273788435904,-13.7830867439208));
#47418=CARTESIAN_POINT('Ctrl Pts',(16.3380758082444,18.3053109799212,-13.7872703577417));
#47419=CARTESIAN_POINT('Ctrl Pts',(16.3094902338593,18.384875816755,-13.7914539715626));
#47420=CARTESIAN_POINT('Ctrl Pts',(16.2849076425234,18.4656499986249,-13.7956375853835));
#47421=CARTESIAN_POINT('Ctrl Pts',(16.260736137924,18.5450734199358,-13.7997512379815));
#47422=CARTESIAN_POINT('Ctrl Pts',(16.2404348481342,18.625665568199,-13.8038648905794));
#47423=CARTESIAN_POINT('Ctrl Pts',(16.2241009663663,18.7070090864265,-13.8079785431774));
#47424=CARTESIAN_POINT('Ctrl Pts',(16.2073503971231,18.7904277283583,-13.8121971376098));
#47425=CARTESIAN_POINT('Ctrl Pts',(16.1947725425285,18.8746360871018,-13.8164157320421));
#47426=CARTESIAN_POINT('Ctrl Pts',(16.1864159534739,18.9591756050623,-13.8206343264745));
#47427=CARTESIAN_POINT('Ctrl Pts',(16.1780593644194,19.0437151230227,-13.8248529209068));
#47428=CARTESIAN_POINT('Ctrl Pts',(16.1739240322153,19.1285852645551,-13.8290715153392));
#47429=CARTESIAN_POINT('Ctrl Pts',(16.1740010575059,19.2133268925441,-13.8332901097715));
#47430=CARTESIAN_POINT('Ctrl Pts',(16.1735504167883,19.2133273021507,-13.8332901097715));
#47431=CARTESIAN_POINT('Ctrl Pts',(16.1718448984259,19.397218647613,-13.8424428639771));
#47432=CARTESIAN_POINT('Ctrl Pts',(16.2739023704358,20.430943821993,-13.8939875537431));
#47433=CARTESIAN_POINT('Ctrl Pts',(17.6781137250704,22.0479692933859,-13.9879241790696));
#47434=CARTESIAN_POINT('Ctrl Pts',(19.6033699085088,21.7705394915115,-14.073242403535));
#47435=CARTESIAN_POINT('Ctrl Pts',(20.2876322249798,21.2509972054334,-14.1161686924399));
#47436=CARTESIAN_POINT('Ctrl Pts',(20.2961055941918,21.2444717899281,-14.1167030457843));
#47437=CARTESIAN_POINT('',(16.1740010826188,19.2086456408846,-13.7667098774927));
#47438=CARTESIAN_POINT('Ctrl Pts',(16.1744182524956,19.2086462806443,-13.7667098902285));
#47439=CARTESIAN_POINT('Ctrl Pts',(16.1802301046829,19.8484613837252,-13.7985275695778));
#47440=CARTESIAN_POINT('Ctrl Pts',(16.7471749375075,21.3499116609599,-13.8727371844876));
#47441=CARTESIAN_POINT('Ctrl Pts',(18.7905373386876,22.0308988273534,-13.967209816535));
#47442=CARTESIAN_POINT('Ctrl Pts',(19.9669551389709,21.4873580195988,-14.0298647692332));
#47443=CARTESIAN_POINT('Ctrl Pts',(20.2909850521016,21.2378231040073,-14.0501277863708));
#47444=CARTESIAN_POINT('Ctrl Pts',(20.2935358855687,21.2411349269503,-13.2501880127039));
#47445=CARTESIAN_POINT('Ctrl Pts',(20.3621095148682,21.1884571298854,-13.2544909997392));
#47446=CARTESIAN_POINT('Ctrl Pts',(20.428092506028,21.1322385438866,-13.2587939867745));
#47447=CARTESIAN_POINT('Ctrl Pts',(20.4911037546367,21.0727696945223,-13.2630969738097));
#47448=CARTESIAN_POINT('Ctrl Pts',(20.5521864281439,21.0151209986183,-13.2672682600163));
#47449=CARTESIAN_POINT('Ctrl Pts',(20.6104762812547,20.9544184654227,-13.2714395462229));
#47450=CARTESIAN_POINT('Ctrl Pts',(20.6656594856219,20.8909677471924,-13.2756108324295));
#47451=CARTESIAN_POINT('Ctrl Pts',(20.7208228005176,20.8275398982622,-13.2797806151954));
#47452=CARTESIAN_POINT('Ctrl Pts',(20.7728813887447,20.7613661781835,-13.2839503979612));
#47453=CARTESIAN_POINT('Ctrl Pts',(20.8215597165041,20.6927875792533,-13.2881201807271));
#47454=CARTESIAN_POINT('Ctrl Pts',(20.8702351016398,20.6242131259259,-13.2922897114279));
#47455=CARTESIAN_POINT('Ctrl Pts',(20.9155303667627,20.5532344582363,-13.2964592421288));
#47456=CARTESIAN_POINT('Ctrl Pts',(20.9572123825738,20.4802228732459,-13.3006287728297));
#47457=CARTESIAN_POINT('Ctrl Pts',(20.9989043820684,20.4071938005081,-13.3047993022172));
#47458=CARTESIAN_POINT('Ctrl Pts',(21.0369811868537,20.3321312436427,-13.3089698316048));
#47459=CARTESIAN_POINT('Ctrl Pts',(21.0712555039942,20.2554312849818,-13.3131403609924));
#47460=CARTESIAN_POINT('Ctrl Pts',(21.1055689017353,20.178643870736,-13.3173156457422));
#47461=CARTESIAN_POINT('Ctrl Pts',(21.13607097399,20.1002157503588,-13.321490930492));
#47462=CARTESIAN_POINT('Ctrl Pts',(21.1626227258789,20.0205626321321,-13.3256662152417));
#47463=CARTESIAN_POINT('Ctrl Pts',(21.1891927332993,19.9408547487803,-13.3298443706889));
#47464=CARTESIAN_POINT('Ctrl Pts',(21.2118068922775,19.8599206339596,-13.334022526136));
#47465=CARTESIAN_POINT('Ctrl Pts',(21.2303768166874,19.7781884952162,-13.3382006815831));
#47466=CARTESIAN_POINT('Ctrl Pts',(21.2489760425118,19.696327391636,-13.342385429726));
#47467=CARTESIAN_POINT('Ctrl Pts',(21.2635182246709,19.6136662038172,-13.346570177869));
#47468=CARTESIAN_POINT('Ctrl Pts',(21.2739665897943,19.5306399892512,-13.350754926012));
#47469=CARTESIAN_POINT('Ctrl Pts',(21.2762176597463,19.5127522322071,-13.3516565178582));
#47470=CARTESIAN_POINT('Ctrl Pts',(21.2782788975167,19.4948475346138,-13.3525581097044));
#47471=CARTESIAN_POINT('Ctrl Pts',(21.2801502518719,19.4769302444118,-13.3534597015506));
#47472=CARTESIAN_POINT('Ctrl Pts',(21.2888359269133,19.3937692119263,-13.3576443359436));
#47473=CARTESIAN_POINT('Ctrl Pts',(21.2934592377886,19.3100274422731,-13.3618289703367));
#47474=CARTESIAN_POINT('Ctrl Pts',(21.2939552539536,19.2261359755289,-13.3660136047297));
#47475=CARTESIAN_POINT('Ctrl Pts',(21.294450564101,19.1423639179039,-13.3701922828137));
#47476=CARTESIAN_POINT('Ctrl Pts',(21.2908302458307,19.0584430425126,-13.3743709608976));
#47477=CARTESIAN_POINT('Ctrl Pts',(21.2830810689264,18.9748100255276,-13.3785496389816));
#47478=CARTESIAN_POINT('Ctrl Pts',(21.2751929935952,18.8896779468192,-13.382803216867));
#47479=CARTESIAN_POINT('Ctrl Pts',(21.2630265340501,18.804844627276,-13.3870567947524));
#47480=CARTESIAN_POINT('Ctrl Pts',(21.2466232879999,18.7207712650195,-13.3913103726379));
#47481=CARTESIAN_POINT('Ctrl Pts',(21.2305380508827,18.6383278289459,-13.3954814866158));
#47482=CARTESIAN_POINT('Ctrl Pts',(21.2103789301822,18.5566156189164,-13.3996526005938));
#47483=CARTESIAN_POINT('Ctrl Pts',(21.1862373001536,18.4760631158151,-13.4038237145717));
#47484=CARTESIAN_POINT('Ctrl Pts',(21.1621037710821,18.3955376428842,-13.4079934288921));
#47485=CARTESIAN_POINT('Ctrl Pts',(21.1339905186921,18.3161715443229,-13.4121631432125));
#47486=CARTESIAN_POINT('Ctrl Pts',(21.1020392245073,18.2383797086247,-13.4163328575329));
#47487=CARTESIAN_POINT('Ctrl Pts',(21.0700890672866,18.1605906410939,-13.4205024234769));
#47488=CARTESIAN_POINT('Ctrl Pts',(21.0343013153839,18.0843761502596,-13.4246719894209));
#47489=CARTESIAN_POINT('Ctrl Pts',(20.9948658827287,18.0101313725834,-13.428841555365));
#47490=CARTESIAN_POINT('Ctrl Pts',(20.9540439489102,17.933276240115,-13.4331577181039));
#47491=CARTESIAN_POINT('Ctrl Pts',(20.9093133043206,17.8585323739429,-13.4374738808428));
#47492=CARTESIAN_POINT('Ctrl Pts',(20.8609355752997,17.7863087848504,-13.4417900435817));
#47493=CARTESIAN_POINT('Ctrl Pts',(20.8141337457132,17.7164378715759,-13.4459656077734));
#47494=CARTESIAN_POINT('Ctrl Pts',(20.7639191093595,17.6489259106341,-13.4501411719651));
#47495=CARTESIAN_POINT('Ctrl Pts',(20.7105706701801,17.5841108255988,-13.4543167361568));
#47496=CARTESIAN_POINT('Ctrl Pts',(20.6545277281616,17.5160220847016,-13.4587031981693));
#47497=CARTESIAN_POINT('Ctrl Pts',(20.5950264806455,17.450910248947,-13.4630896601819));
#47498=CARTESIAN_POINT('Ctrl Pts',(20.5324338669329,17.3891230485379,-13.4674761221944));
#47499=CARTESIAN_POINT('Ctrl Pts',(20.4698412532203,17.3273358481288,-13.4718625842069));
#47500=CARTESIAN_POINT('Ctrl Pts',(20.4041577572906,17.2688736120053,-13.4762490462195));
#47501=CARTESIAN_POINT('Ctrl Pts',(20.3357880909559,17.2140335727229,-13.480635508232));
#47502=CARTESIAN_POINT('Ctrl Pts',(20.2705642143173,17.1617168049402,-13.4848201426251));
#47503=CARTESIAN_POINT('Ctrl Pts',(20.2026531489501,17.1125015005239,-13.4890047770181));
#47504=CARTESIAN_POINT('Ctrl Pts',(20.1323821856731,17.0666755696043,-13.4931894114112));
#47505=CARTESIAN_POINT('Ctrl Pts',(20.0622112444146,17.0209148662252,-13.4973680894951));
#47506=CARTESIAN_POINT('Ctrl Pts',(19.9896874593622,16.9785342027988,-13.5015467675791));
#47507=CARTESIAN_POINT('Ctrl Pts',(19.9151708448062,16.9397810683732,-13.505725445663));
#47508=CARTESIAN_POINT('Ctrl Pts',(19.8393185734883,16.9003333118644,-13.5099790235484));
#47509=CARTESIAN_POINT('Ctrl Pts',(19.7614017031198,16.8646447120803,-13.5142326014339));
#47510=CARTESIAN_POINT('Ctrl Pts',(19.6818305443853,16.8329299297266,-13.5184861793193));
#47511=CARTESIAN_POINT('Ctrl Pts',(19.6038020278331,16.801830000315,-13.5226572932973));
#47512=CARTESIAN_POINT('Ctrl Pts',(19.5241832407486,16.7745513610798,-13.5268284072752));
#47513=CARTESIAN_POINT('Ctrl Pts',(19.4433839268982,16.7512491093083,-13.5309995212532));
#47514=CARTESIAN_POINT('Ctrl Pts',(19.3626117260379,16.7279546768325,-13.5351692355735));
#47515=CARTESIAN_POINT('Ctrl Pts',(19.2806602267965,16.7086341092198,-13.5393389498939));
#47516=CARTESIAN_POINT('Ctrl Pts',(19.1979549742612,16.6933928460027,-13.5435086642143));
#47517=CARTESIAN_POINT('Ctrl Pts',(19.1152526647337,16.6781521251352,-13.5476782301583));
#47518=CARTESIAN_POINT('Ctrl Pts',(19.0317971078103,16.6669905025844,-13.5518477961024));
#47519=CARTESIAN_POINT('Ctrl Pts',(18.9480233475313,16.6599621706624,-13.5560173620464));
#47520=CARTESIAN_POINT('Ctrl Pts',(18.861304205187,16.6526867312604,-13.5603335247853));
#47521=CARTESIAN_POINT('Ctrl Pts',(18.7742445926769,16.6498406874529,-13.5646496875243));
#47522=CARTESIAN_POINT('Ctrl Pts',(18.687330036718,16.6514254426707,-13.5689658502632));
#47523=CARTESIAN_POINT('Ctrl Pts',(18.6032467132777,16.6529585746541,-13.5731414144549));
#47524=CARTESIAN_POINT('Ctrl Pts',(18.5192996078628,16.6586381931969,-13.5773169786466));
#47525=CARTESIAN_POINT('Ctrl Pts',(18.435923880263,16.6684126117589,-13.5814925428382));
#47526=CARTESIAN_POINT('Ctrl Pts',(18.3483370428692,16.678680712966,-13.5858790048508));
#47527=CARTESIAN_POINT('Ctrl Pts',(18.2613813964209,16.6934680441002,-13.5902654668633));
#47528=CARTESIAN_POINT('Ctrl Pts',(18.1755479442734,16.7126542870422,-13.5946519288759));
#47529=CARTESIAN_POINT('Ctrl Pts',(18.089714492126,16.7318405299841,-13.5990383908884));
#47530=CARTESIAN_POINT('Ctrl Pts',(18.0050037728349,16.7554254558327,-13.6034248529009));
#47531=CARTESIAN_POINT('Ctrl Pts',(17.921884774769,16.783229652346,-13.6078113149135));
#47532=CARTESIAN_POINT('Ctrl Pts',(17.842590205016,16.809754536562,-13.6119959493065));
#47533=CARTESIAN_POINT('Ctrl Pts',(17.7644489508447,16.8402176845382,-13.6161805836996));
#47534=CARTESIAN_POINT('Ctrl Pts',(17.6878802554244,16.8744997367839,-13.6203652180926));
#47535=CARTESIAN_POINT('Ctrl Pts',(17.6114205460648,16.9087329927714,-13.6245438961766));
#47536=CARTESIAN_POINT('Ctrl Pts',(17.536529365682,16.9467741695629,-13.6287225742605));
#47537=CARTESIAN_POINT('Ctrl Pts',(17.4636096823067,16.9884545132414,-13.6329012523445));
#47538=CARTESIAN_POINT('Ctrl Pts',(17.3893829660134,17.0308819471251,-13.6371548302299));
#47539=CARTESIAN_POINT('Ctrl Pts',(17.3171995773182,17.0770801423177,-13.6414084081153));
#47540=CARTESIAN_POINT('Ctrl Pts',(17.2474621052952,17.1268202842349,-13.6456619860008));
#47541=CARTESIAN_POINT('Ctrl Pts',(17.1790766302489,17.1755961164411,-13.6498330999787));
#47542=CARTESIAN_POINT('Ctrl Pts',(17.1130434722312,17.2277775063952,-13.6540042139567));
#47543=CARTESIAN_POINT('Ctrl Pts',(17.0497148300457,17.283103875653,-13.6581753279346));
#47544=CARTESIAN_POINT('Ctrl Pts',(16.9864074383977,17.3384116796134,-13.662345042255));
#47545=CARTESIAN_POINT('Ctrl Pts',(16.9258031063753,17.3968620645642,-13.6665147565754));
#47546=CARTESIAN_POINT('Ctrl Pts',(16.8682208314237,17.4581542868504,-13.6706844708957));
#47547=CARTESIAN_POINT('Ctrl Pts',(16.8106406054967,17.5194443280963,-13.6748540368398));
#47548=CARTESIAN_POINT('Ctrl Pts',(16.7560825371937,17.5835756697509,-13.6790236027838));
#47549=CARTESIAN_POINT('Ctrl Pts',(16.7048276747609,17.650211841894,-13.6831931687278));
#47550=CARTESIAN_POINT('Ctrl Pts',(16.6517707545947,17.7191908596451,-13.6875093314668));
#47551=CARTESIAN_POINT('Ctrl Pts',(16.6022539651133,17.7908537067501,-13.6918254942057));
#47552=CARTESIAN_POINT('Ctrl Pts',(16.5565412927829,17.8647928917271,-13.6961416569446));
#47553=CARTESIAN_POINT('Ctrl Pts',(16.5123177059456,17.9363235155304,-13.7003172211363));
#47554=CARTESIAN_POINT('Ctrl Pts',(16.4716543903427,18.0099840160617,-13.704492785328));
#47555=CARTESIAN_POINT('Ctrl Pts',(16.4347434295141,18.0853805158593,-13.7086683495197));
#47556=CARTESIAN_POINT('Ctrl Pts',(16.3959681838015,18.1645851136235,-13.7130548115322));
#47557=CARTESIAN_POINT('Ctrl Pts',(16.3613345469612,18.2457051531361,-13.7174412735447));
#47558=CARTESIAN_POINT('Ctrl Pts',(16.3310071212994,18.3282626523624,-13.7218277355573));
#47559=CARTESIAN_POINT('Ctrl Pts',(16.3006796956376,18.4108201515888,-13.7262141975698));
#47560=CARTESIAN_POINT('Ctrl Pts',(16.2746585801944,18.494814533789,-13.7306006595824));
#47561=CARTESIAN_POINT('Ctrl Pts',(16.253046772176,18.5797543415202,-13.7349871215949));
#47562=CARTESIAN_POINT('Ctrl Pts',(16.2263033450825,18.6848626949471,-13.7404151277539));
#47563=CARTESIAN_POINT('Ctrl Pts',(16.2062281520531,18.7917315462651,-13.7458431339129));
#47564=CARTESIAN_POINT('Ctrl Pts',(16.1930065418683,18.8996284442475,-13.7512711400719));
#47565=CARTESIAN_POINT('Ctrl Pts',(16.180471247327,19.0019245622985,-13.7564173858788));
#47566=CARTESIAN_POINT('Ctrl Pts',(16.1740962693074,19.1051449394228,-13.7615636316857));
#47567=CARTESIAN_POINT('Ctrl Pts',(16.1740010826188,19.2086456408846,-13.7667098774927));
#47568=CARTESIAN_POINT('Origin',(18.734,19.211,1.76670989022852));
#47569=CARTESIAN_POINT('',(20.2954167287344,21.2436206075649,-12.4500366863435));
#47570=CARTESIAN_POINT('',(20.2935358855687,21.2411349269503,-12.5167193513141));
#47571=CARTESIAN_POINT('',(20.2935358855687,21.2411349269503,1.76670989022852));
#47572=CARTESIAN_POINT('',(16.174000001606,19.2109093211998,-13.0332901097364));
#47573=CARTESIAN_POINT('Ctrl Pts',(20.2935358855687,21.2411349269503,-12.5167193513141));
#47574=CARTESIAN_POINT('Ctrl Pts',(20.3602126462826,21.1899142914712,-12.5208888671653));
#47575=CARTESIAN_POINT('Ctrl Pts',(20.4243799329773,21.1353926325048,-12.5250583830165));
#47576=CARTESIAN_POINT('Ctrl Pts',(20.4857025030192,21.0778525225407,-12.5292278988677));
#47577=CARTESIAN_POINT('Ctrl Pts',(20.5470295679466,21.0203081949416,-12.5333977203404));
#47578=CARTESIAN_POINT('Ctrl Pts',(20.6055111676078,20.959745292768,-12.5375675418131));
#47579=CARTESIAN_POINT('Ctrl Pts',(20.6608480428545,20.8964840906243,-12.5417373632858));
#47580=CARTESIAN_POINT('Ctrl Pts',(20.7162427463173,20.8331567791739,-12.5459115423109));
#47581=CARTESIAN_POINT('Ctrl Pts',(20.7684858595219,20.7671258839871,-12.5500857213361));
#47582=CARTESIAN_POINT('Ctrl Pts',(20.8173179955917,20.6987453173322,-12.5542599003612));
#47583=CARTESIAN_POINT('Ctrl Pts',(20.8661764272834,20.630327928419,-12.5584363271405));
#47584=CARTESIAN_POINT('Ctrl Pts',(20.9116199755333,20.5595587357766,-12.5626127539197));
#47585=CARTESIAN_POINT('Ctrl Pts',(20.9534335841905,20.4868191742436,-12.5667891806989));
#47586=CARTESIAN_POINT('Ctrl Pts',(20.9953200408688,20.4139528852338,-12.5709728836841));
#47587=CARTESIAN_POINT('Ctrl Pts',(21.0335637164752,20.3391097806619,-12.5751565866692));
#47588=CARTESIAN_POINT('Ctrl Pts',(21.067996451488,20.2626941401574,-12.5793402896544));
#47589=CARTESIAN_POINT('Ctrl Pts',(21.094470322618,20.2039413916964,-12.5825569616276));
#47590=CARTESIAN_POINT('Ctrl Pts',(21.1186923490915,20.1442595308903,-12.5857736336007));
#47591=CARTESIAN_POINT('Ctrl Pts',(21.1406062076889,20.0838382216157,-12.5889903055739));
#47592=CARTESIAN_POINT('Ctrl Pts',(21.1691143947643,20.0052349039716,-12.5931749399669));
#47593=CARTESIAN_POINT('Ctrl Pts',(21.193820633909,19.9250871608006,-12.59735957436));
#47594=CARTESIAN_POINT('Ctrl Pts',(21.2145578396958,19.8437976010731,-12.601544208753));
#47595=CARTESIAN_POINT('Ctrl Pts',(21.2352655286368,19.7626237469725,-12.605722886837));
#47596=CARTESIAN_POINT('Ctrl Pts',(21.2520152930198,19.6803117464873,-12.6099015649209));
#47597=CARTESIAN_POINT('Ctrl Pts',(21.2646888572062,19.5972821611367,-12.6140802430048));
#47598=CARTESIAN_POINT('Ctrl Pts',(21.2775895859223,19.5127643301408,-12.6183338208903));
#47599=CARTESIAN_POINT('Ctrl Pts',(21.2862663809328,19.4275033890779,-12.6225873987757));
#47600=CARTESIAN_POINT('Ctrl Pts',(21.290648251397,19.3419569342516,-12.6268409766611));
#47601=CARTESIAN_POINT('Ctrl Pts',(21.2949451707517,19.2580689643825,-12.6310120906391));
#47602=CARTESIAN_POINT('Ctrl Pts',(21.2951121858363,19.1739069330306,-12.635183204617));
#47603=CARTESIAN_POINT('Ctrl Pts',(21.2911345092732,19.089908705993,-12.639354318595));
#47604=CARTESIAN_POINT('Ctrl Pts',(21.2871581674578,19.0059386653716,-12.6435240329154));
#47605=CARTESIAN_POINT('Ctrl Pts',(21.2790399178705,18.9221327790365,-12.6476937472357));
#47606=CARTESIAN_POINT('Ctrl Pts',(21.2668170738606,18.8389278694117,-12.6518634615561));
#47607=CARTESIAN_POINT('Ctrl Pts',(21.2545946647918,18.7557259205746,-12.6560330275001));
#47608=CARTESIAN_POINT('Ctrl Pts',(21.2382680194081,18.6731253609524,-12.6602025934442));
#47609=CARTESIAN_POINT('Ctrl Pts',(21.2179260255781,18.5915554912215,-12.6643721593882));
#47610=CARTESIAN_POINT('Ctrl Pts',(21.1968688323395,18.5071177254981,-12.6686883221272));
#47611=CARTESIAN_POINT('Ctrl Pts',(21.1715088054104,18.4237849880539,-12.6730044848661));
#47612=CARTESIAN_POINT('Ctrl Pts',(21.142001073276,18.342017358573,-12.677320647605));
#47613=CARTESIAN_POINT('Ctrl Pts',(21.1134545524123,18.2629133010222,-12.6814962117967));
#47614=CARTESIAN_POINT('Ctrl Pts',(21.0810266246881,18.1852743669889,-12.6856717759884));
#47615=CARTESIAN_POINT('Ctrl Pts',(21.0449064462661,18.1094958481215,-12.68984734018));
#47616=CARTESIAN_POINT('Ctrl Pts',(21.0069619234994,18.0298899364119,-12.6942338021926));
#47617=CARTESIAN_POINT('Ctrl Pts',(20.964942634636,17.9523378315096,-12.6986202642051));
#47618=CARTESIAN_POINT('Ctrl Pts',(20.9191207015649,17.8772655738144,-12.7030067262177));
#47619=CARTESIAN_POINT('Ctrl Pts',(20.8732987684938,17.8021933161193,-12.7073931882302));
#47620=CARTESIAN_POINT('Ctrl Pts',(20.8236745814509,17.7296013416973,-12.7117796502428));
#47621=CARTESIAN_POINT('Ctrl Pts',(20.7705691100603,17.6598758076968,-12.7161661122553));
#47622=CARTESIAN_POINT('Ctrl Pts',(20.7199071001298,17.593358448874,-12.7203507466484));
#47623=CARTESIAN_POINT('Ctrl Pts',(20.6658885504365,17.5292019583443,-12.7245353810414));
#47624=CARTESIAN_POINT('Ctrl Pts',(20.6087615512377,17.4677647531096,-12.7287200154345));
#47625=CARTESIAN_POINT('Ctrl Pts',(20.5517158652512,17.4064149961321,-12.7328986935184));
#47626=CARTESIAN_POINT('Ctrl Pts',(20.4915708287755,17.3477771703014,-12.7370773716023));
#47627=CARTESIAN_POINT('Ctrl Pts',(20.4286160471331,17.2921783686859,-12.7412560496863));
#47628=CARTESIAN_POINT('Ctrl Pts',(20.3645328462747,17.2355829985097,-12.7455096275717));
#47629=CARTESIAN_POINT('Ctrl Pts',(20.2975384722481,17.1821370567428,-12.7497632054572));
#47630=CARTESIAN_POINT('Ctrl Pts',(20.2279792651328,17.1321479236479,-12.7540167833426));
#47631=CARTESIAN_POINT('Ctrl Pts',(20.159768598981,17.0831279274438,-12.7581878973205));
#47632=CARTESIAN_POINT('Ctrl Pts',(20.0890920516418,17.0374321828769,-12.7623590112985));
#47633=CARTESIAN_POINT('Ctrl Pts',(20.0163097948298,16.9953101322424,-12.7665301252764));
#47634=CARTESIAN_POINT('Ctrl Pts',(19.9435519608069,16.9532022160688,-12.7706998395968));
#47635=CARTESIAN_POINT('Ctrl Pts',(19.8686902184412,16.9146658424621,-12.7748695539172));
#47636=CARTESIAN_POINT('Ctrl Pts',(19.7921120632711,16.8799060804935,-12.7790392682375));
#47637=CARTESIAN_POINT('Ctrl Pts',(19.7155366330805,16.8451475554265,-12.7832088341816));
#47638=CARTESIAN_POINT('Ctrl Pts',(19.6372453307736,16.8141655641666,-12.7873784001256));
#47639=CARTESIAN_POINT('Ctrl Pts',(19.557647243598,16.7871177383971,-12.7915479660697));
#47640=CARTESIAN_POINT('Ctrl Pts',(19.4752505858722,16.7591189444405,-12.7958641288086));
#47641=CARTESIAN_POINT('Ctrl Pts',(19.3914540397877,16.7353362835285,-12.8001802915475));
#47642=CARTESIAN_POINT('Ctrl Pts',(19.3067284276563,16.7158883495614,-12.8044964542864));
#47643=CARTESIAN_POINT('Ctrl Pts',(19.2247627434286,16.6970739299978,-12.8086720184781));
#47644=CARTESIAN_POINT('Ctrl Pts',(19.1419280643013,16.6823162029296,-12.8128475826698));
#47645=CARTESIAN_POINT('Ctrl Pts',(19.0586591546378,16.6716700818307,-12.8170231468614));
#47646=CARTESIAN_POINT('Ctrl Pts',(18.9711845303002,16.6604862504638,-12.821409608874));
#47647=CARTESIAN_POINT('Ctrl Pts',(18.8832312388615,16.6538403392096,-12.8257960708865));
#47648=CARTESIAN_POINT('Ctrl Pts',(18.7953048072929,16.6517341442119,-12.830182532899));
#47649=CARTESIAN_POINT('Ctrl Pts',(18.7073783757243,16.6496279492142,-12.8345689949116));
#47650=CARTESIAN_POINT('Ctrl Pts',(18.6194793819155,16.6520613783803,-12.8389554569241));
#47651=CARTESIAN_POINT('Ctrl Pts',(18.5321062576876,16.6589735665916,-12.8433419189367));
#47652=CARTESIAN_POINT('Ctrl Pts',(18.4487533004234,16.665567714777,-12.8475265533297));
#47653=CARTESIAN_POINT('Ctrl Pts',(18.3655686284663,16.6762620749485,-12.8517111877228));
#47654=CARTESIAN_POINT('Ctrl Pts',(18.2829879003453,16.6910420467863,-12.8558958221158));
#47655=CARTESIAN_POINT('Ctrl Pts',(18.2005247156695,16.7058009811635,-12.8600745001997));
#47656=CARTESIAN_POINT('Ctrl Pts',(18.1186642162797,16.7246338957133,-12.8642531782837));
#47657=CARTESIAN_POINT('Ctrl Pts',(18.0378381935513,16.7474743274644,-12.8684318563676));
#47658=CARTESIAN_POINT('Ctrl Pts',(17.9555634224539,16.7707241575396,-12.872685434253));
#47659=CARTESIAN_POINT('Ctrl Pts',(17.8743610594197,16.7981265494104,-12.8769390121385));
#47660=CARTESIAN_POINT('Ctrl Pts',(17.7946770299218,16.8295566649858,-12.8811925900239));
#47661=CARTESIAN_POINT('Ctrl Pts',(17.7165378308264,16.8603774464399,-12.8853637040019));
#47662=CARTESIAN_POINT('Ctrl Pts',(17.639859066566,16.8950709981002,-12.8895348179798));
#47663=CARTESIAN_POINT('Ctrl Pts',(17.5650454327538,16.9334694909367,-12.8937059319578));
#47664=CARTESIAN_POINT('Ctrl Pts',(17.4902569033788,16.9718550987881,-12.8978756462781));
#47665=CARTESIAN_POINT('Ctrl Pts',(17.4173326704116,17.0139429688568,-12.9020453605985));
#47666=CARTESIAN_POINT('Ctrl Pts',(17.3466549084735,17.0595182787164,-12.9062150749189));
#47667=CARTESIAN_POINT('Ctrl Pts',(17.2759796615535,17.105091966811,-12.9103846408629));
#47668=CARTESIAN_POINT('Ctrl Pts',(17.2075511128834,17.154152597935,-12.914554206807));
#47669=CARTESIAN_POINT('Ctrl Pts',(17.1417232369313,17.2064415174929,-12.918723772751));
#47670=CARTESIAN_POINT('Ctrl Pts',(17.0735809340681,17.260568850957,-12.92303993549));
#47671=CARTESIAN_POINT('Ctrl Pts',(17.0082259988603,17.3181553818453,-12.9273560982289));
#47672=CARTESIAN_POINT('Ctrl Pts',(16.9460129971978,17.3788694157319,-12.9316722609678));
#47673=CARTESIAN_POINT('Ctrl Pts',(16.8858265775208,17.4376056963507,-12.9358478251595));
#47674=CARTESIAN_POINT('Ctrl Pts',(16.8285808237897,17.499268474865,-12.9400233893512));
#47675=CARTESIAN_POINT('Ctrl Pts',(16.7745572392495,17.5635219068702,-12.9441989535429));
#47676=CARTESIAN_POINT('Ctrl Pts',(16.7178050518831,17.631020626978,-12.9485854155554));
#47677=CARTESIAN_POINT('Ctrl Pts',(16.6646094437668,17.7013781204557,-12.9529718775679));
#47678=CARTESIAN_POINT('Ctrl Pts',(16.6152455573348,17.7741702913405,-12.9573583395805));
#47679=CARTESIAN_POINT('Ctrl Pts',(16.5658816709029,17.8469624622252,-12.961744801593));
#47680=CARTESIAN_POINT('Ctrl Pts',(16.5203497415206,17.9221887747551,-12.9661312636056));
#47681=CARTESIAN_POINT('Ctrl Pts',(16.4788683829465,17.9993971815129,-12.9705177256181));
#47682=CARTESIAN_POINT('Ctrl Pts',(16.4371381237559,18.0770688619124,-12.9749305077209));
#47683=CARTESIAN_POINT('Ctrl Pts',(16.3993648293881,18.1570094498413,-12.9793432898236));
#47684=CARTESIAN_POINT('Ctrl Pts',(16.3657873879884,18.2388019624021,-12.9837560719264));
#47685=CARTESIAN_POINT('Ctrl Pts',(16.3323070847556,18.3203578525641,-12.9881560880307));
#47686=CARTESIAN_POINT('Ctrl Pts',(16.3029985969533,18.4037546379833,-12.992556104135));
#47687=CARTESIAN_POINT('Ctrl Pts',(16.2780542372553,18.4885524860197,-12.9969561202393));
#47688=CARTESIAN_POINT('Ctrl Pts',(16.2531532512187,18.5732028861683,-13.0013484855236));
#47689=CARTESIAN_POINT('Ctrl Pts',(16.2326014031163,18.6592491335653,-13.0057408508078));
#47690=CARTESIAN_POINT('Ctrl Pts',(16.2165427462274,18.7462323425329,-13.010133216092));
#47691=CARTESIAN_POINT('Ctrl Pts',(16.2005210016679,18.833015612434,-13.0145154851125));
#47692=CARTESIAN_POINT('Ctrl Pts',(16.1889719431304,18.9207311752712,-13.018897754133));
#47693=CARTESIAN_POINT('Ctrl Pts',(16.1819893075699,19.0089073833058,-13.0232800231536));
#47694=CARTESIAN_POINT('Ctrl Pts',(16.176672671659,19.0760454703589,-13.0266167186812));
#47695=CARTESIAN_POINT('Ctrl Pts',(16.1740023911013,19.1434502453368,-13.0299534142088));
#47696=CARTESIAN_POINT('Ctrl Pts',(16.174000001606,19.2109093211998,-13.0332901097364));
#47697=CARTESIAN_POINT('Ctrl Pts',(16.174000001606,19.2109093219104,-13.0332901097715));
#47698=CARTESIAN_POINT('Ctrl Pts',(16.1739968821085,19.2989781543512,-13.0376462156856));
#47699=CARTESIAN_POINT('Ctrl Pts',(16.1785426714359,19.3869643923453,-13.0420023215996));
#47700=CARTESIAN_POINT('Ctrl Pts',(16.1875860737585,19.4743934627951,-13.0463584275137));
#47701=CARTESIAN_POINT('Ctrl Pts',(16.1966529338893,19.5620493167382,-13.0507258327921));
#47702=CARTESIAN_POINT('Ctrl Pts',(16.2102406836426,19.6491447181138,-13.0550932380704));
#47703=CARTESIAN_POINT('Ctrl Pts',(16.2282463851319,19.7352125728895,-13.0594606433488));
#47704=CARTESIAN_POINT('Ctrl Pts',(16.2462755658189,19.8213926590147,-13.0638337436661));
#47705=CARTESIAN_POINT('Ctrl Pts',(16.2687340840994,19.9065421429603,-13.0682068439834));
#47706=CARTESIAN_POINT('Ctrl Pts',(16.2954690366782,19.9902090482795,-13.0725799443008));
#47707=CARTESIAN_POINT('Ctrl Pts',(16.3222767415773,20.0741036316347,-13.0769649448896));
#47708=CARTESIAN_POINT('Ctrl Pts',(16.3533840099471,20.1565071961889,-13.0813499454785));
#47709=CARTESIAN_POINT('Ctrl Pts',(16.3885892814888,20.2369866283206,-13.0857349460673));
#47710=CARTESIAN_POINT('Ctrl Pts',(16.4205927188907,20.310146651112,-13.0897211414781));
#47711=CARTESIAN_POINT('Ctrl Pts',(16.4559819492917,20.3817167133684,-13.0937073368888));
#47712=CARTESIAN_POINT('Ctrl Pts',(16.4945737975983,20.4513911818441,-13.0976935322996));
#47713=CARTESIAN_POINT('Ctrl Pts',(16.5350868078939,20.524534153289,-13.1018781666926));
#47714=CARTESIAN_POINT('Ctrl Pts',(16.5792624158945,20.5958263313022,-13.1060628010857));
#47715=CARTESIAN_POINT('Ctrl Pts',(16.6269069559,20.6648771968449,-13.1102474354787));
#47716=CARTESIAN_POINT('Ctrl Pts',(16.6744836798,20.7338297770272,-13.1144261135626));
#47717=CARTESIAN_POINT('Ctrl Pts',(16.7255192690591,20.8005470061347,-13.1186047916466));
#47718=CARTESIAN_POINT('Ctrl Pts',(16.7797744504213,20.8646633579341,-13.1227834697305));
#47719=CARTESIAN_POINT('Ctrl Pts',(16.8350021169169,20.9299289492599,-13.127037047616));
#47720=CARTESIAN_POINT('Ctrl Pts',(16.8935656995718,20.9924990829437,-13.1312906255014));
#47721=CARTESIAN_POINT('Ctrl Pts',(16.9551669364597,21.0520195360332,-13.1355442033868));
#47722=CARTESIAN_POINT('Ctrl Pts',(17.0155739131657,21.110386068995,-13.1397153173648));
#47723=CARTESIAN_POINT('Ctrl Pts',(17.0789014673909,21.1658197797781,-13.1438864313427));
#47724=CARTESIAN_POINT('Ctrl Pts',(17.1448292745178,21.2180217749866,-13.1480575453207));
#47725=CARTESIAN_POINT('Ctrl Pts',(17.2107349589323,21.2702062533115,-13.1522272596411));
#47726=CARTESIAN_POINT('Ctrl Pts',(17.279238803008,21.3191608844269,-13.1563969739614));
#47727=CARTESIAN_POINT('Ctrl Pts',(17.3499870301186,21.364626731632,-13.1605666882818));
#47728=CARTESIAN_POINT('Ctrl Pts',(17.4207327397037,21.4100909609672,-13.1647362542259));
#47729=CARTESIAN_POINT('Ctrl Pts',(17.493722286064,21.4520664052353,-13.1689058201699));
#47730=CARTESIAN_POINT('Ctrl Pts',(17.5685736694553,21.490337945122,-13.1730753861139));
#47731=CARTESIAN_POINT('Ctrl Pts',(17.6460567351475,21.5299550651381,-13.1773915488529));
#47732=CARTESIAN_POINT('Ctrl Pts',(17.7255345286225,21.5656027360313,-13.1817077115918));
#47733=CARTESIAN_POINT('Ctrl Pts',(17.8065583197873,21.5970955407955,-13.1860238743307));
#47734=CARTESIAN_POINT('Ctrl Pts',(17.8849427694771,21.627562470757,-13.1901994385224));
#47735=CARTESIAN_POINT('Ctrl Pts',(17.9647735800336,21.654140963194,-13.1943750027141));
#47736=CARTESIAN_POINT('Ctrl Pts',(18.0456284938942,21.6767138255648,-13.1985505669057));
#47737=CARTESIAN_POINT('Ctrl Pts',(18.1305671972396,21.7004267895521,-13.2029370289183));
#47738=CARTESIAN_POINT('Ctrl Pts',(18.2166356079045,21.7197187126534,-13.2073234909308));
#47739=CARTESIAN_POINT('Ctrl Pts',(18.3033337697291,21.7345147311051,-13.2117099529434));
#47740=CARTESIAN_POINT('Ctrl Pts',(18.3900319315536,21.7493107495567,-13.2160964149559));
#47741=CARTESIAN_POINT('Ctrl Pts',(18.4773592594052,21.7596108709354,-13.2204828769685));
#47742=CARTESIAN_POINT('Ctrl Pts',(18.5648137584886,21.7654032601927,-13.224869338981));
#47743=CARTESIAN_POINT('Ctrl Pts',(18.6482240610122,21.7709277894662,-13.2290529559168));
#47744=CARTESIAN_POINT('Ctrl Pts',(18.7320604262274,21.7723728408952,-13.2332365728525));
#47745=CARTESIAN_POINT('Ctrl Pts',(18.8158899787628,21.7696899052793,-13.2374201897883));
#47746=CARTESIAN_POINT('Ctrl Pts',(18.8996093084477,21.7670104973074,-13.2415983059171));
#47747=CARTESIAN_POINT('Ctrl Pts',(18.9833213878538,21.7602138920977,-13.245776422046));
#47748=CARTESIAN_POINT('Ctrl Pts',(19.0665895300205,21.7493034106507,-13.2499545381748));
#47749=CARTESIAN_POINT('Ctrl Pts',(19.1497731758391,21.7384040006148,-13.2541284145603));
#47750=CARTESIAN_POINT('Ctrl Pts',(19.2325133255147,21.7233990640619,-13.2583022909457));
#47751=CARTESIAN_POINT('Ctrl Pts',(19.3143759725405,21.704343885327,-13.2624761673311));
#47752=CARTESIAN_POINT('Ctrl Pts',(19.3961801113252,21.6853023255629,-13.2666470605958));
#47753=CARTESIAN_POINT('Ctrl Pts',(19.4771075468217,21.6622163790719,-13.2708179538604));
#47754=CARTESIAN_POINT('Ctrl Pts',(19.5567334109213,21.6351925943608,-13.274988847125));
#47755=CARTESIAN_POINT('Ctrl Pts',(19.6363403165266,21.608175243869,-13.2791587473222));
#47756=CARTESIAN_POINT('Ctrl Pts',(19.7146458288504,21.5772220585841,-13.2833286475194));
#47757=CARTESIAN_POINT('Ctrl Pts',(19.7912403187455,21.542489418466,-13.2874985477165));
#47758=CARTESIAN_POINT('Ctrl Pts',(19.8678247271476,21.5077613499152,-13.2916678990645));
#47759=CARTESIAN_POINT('Ctrl Pts',(19.9426981444001,21.4692550109384,-13.2958372504126));
#47760=CARTESIAN_POINT('Ctrl Pts',(20.0154725000694,21.4271742331247,-13.3000066017606));
#47761=CARTESIAN_POINT('Ctrl Pts',(20.0882810786145,21.3850736664003,-13.3041779137882));
#47762=CARTESIAN_POINT('Ctrl Pts',(20.1589882301688,21.3393955415644,-13.3083492258158));
#47763=CARTESIAN_POINT('Ctrl Pts',(20.2272328428135,21.2903882939805,-13.3125205378434));
#47764=CARTESIAN_POINT('Ctrl Pts',(20.2496021795281,21.2743246139305,-13.3138878176868));
#47765=CARTESIAN_POINT('Ctrl Pts',(20.2717071834519,21.257903587907,-13.3152550975302));
#47766=CARTESIAN_POINT('Ctrl Pts',(20.2935358855687,21.2411349269503,-13.3166223773735));
#47767=CARTESIAN_POINT('',(16.1736697067219,19.2116425106688,-12.9667098340815));
#47768=CARTESIAN_POINT('Ctrl Pts',(16.1740000808904,19.2116435515775,-12.9667098902285));
#47769=CARTESIAN_POINT('Ctrl Pts',(16.1740088273484,19.2464363059256,-12.9684506873211));
#47770=CARTESIAN_POINT('Ctrl Pts',(16.1747268399112,19.281219269613,-12.9701914844137));
#47771=CARTESIAN_POINT('Ctrl Pts',(16.1761531171477,19.3159729673894,-12.9719322815063));
#47772=CARTESIAN_POINT('Ctrl Pts',(16.1795816894971,19.3995160291397,-12.9761169158993));
#47773=CARTESIAN_POINT('Ctrl Pts',(16.1871139062631,19.4830464110296,-12.9803015502924));
#47774=CARTESIAN_POINT('Ctrl Pts',(16.1987516982625,19.5661282142232,-12.9844861846854));
#47775=CARTESIAN_POINT('Ctrl Pts',(16.2103729253056,19.6490917607534,-12.9886648627694));
#47776=CARTESIAN_POINT('Ctrl Pts',(16.2260880567289,19.7316075451534,-12.9928435408533));
#47777=CARTESIAN_POINT('Ctrl Pts',(16.2458470513545,19.8132415662726,-12.9970222189372));
#47778=CARTESIAN_POINT('Ctrl Pts',(16.2659602117582,19.896338818551,-13.0012757968227));
#47779=CARTESIAN_POINT('Ctrl Pts',(16.2902636140325,19.9785219036749,-13.0055293747081));
#47780=CARTESIAN_POINT('Ctrl Pts',(16.3186494198466,20.0593404829151,-13.0097829525936));
#47781=CARTESIAN_POINT('Ctrl Pts',(16.3464849114246,20.1385922362921,-13.0139540665715));
#47782=CARTESIAN_POINT('Ctrl Pts',(16.3782457689157,20.2165314648406,-13.0181251805495));
#47783=CARTESIAN_POINT('Ctrl Pts',(16.4137796304916,20.2927473997743,-13.0222962945274));
#47784=CARTESIAN_POINT('Ctrl Pts',(16.4493015683371,20.3689377597149,-13.0264660088478));
#47785=CARTESIAN_POINT('Ctrl Pts',(16.4885938016079,20.4434055578922,-13.0306357231682));
#47786=CARTESIAN_POINT('Ctrl Pts',(16.5314561548597,20.5157607482732,-13.0348054374885));
#47787=CARTESIAN_POINT('Ctrl Pts',(16.574316982885,20.5881133639461,-13.0389750034326));
#47788=CARTESIAN_POINT('Ctrl Pts',(16.6207474431038,20.6583531259277,-13.0431445693766));
#47789=CARTESIAN_POINT('Ctrl Pts',(16.6705024900496,20.7261165058927,-13.0473141353206));
#47790=CARTESIAN_POINT('Ctrl Pts',(16.7220068630667,20.7962623627024,-13.0516302980596));
#47791=CARTESIAN_POINT('Ctrl Pts',(16.7770736453881,20.8637540331555,-13.0559464607985));
#47792=CARTESIAN_POINT('Ctrl Pts',(16.8353848266791,20.9282246281822,-13.0602626235374));
#47793=CARTESIAN_POINT('Ctrl Pts',(16.8917965273727,20.9905951003569,-13.0644381877291));
#47794=CARTESIAN_POINT('Ctrl Pts',(16.951244134227,21.0501379976127,-13.0686137519208));
#47795=CARTESIAN_POINT('Ctrl Pts',(17.0134027193005,21.1065592836019,-13.0727893161124));
#47796=CARTESIAN_POINT('Ctrl Pts',(17.0787007867382,21.1658302746177,-13.077175778125));
#47797=CARTESIAN_POINT('Ctrl Pts',(17.1469904406111,21.2216556522274,-13.0815622401375));
#47798=CARTESIAN_POINT('Ctrl Pts',(17.2178583236868,21.273744389726,-13.0859487021501));
#47799=CARTESIAN_POINT('Ctrl Pts',(17.2887262067624,21.3258331272246,-13.0903351641627));
#47800=CARTESIAN_POINT('Ctrl Pts',(17.3621717925896,21.3741849690991,-13.0947216261752));
#47801=CARTESIAN_POINT('Ctrl Pts',(17.4377516489582,21.4185643167123,-13.0991080881878));
#47802=CARTESIAN_POINT('Ctrl Pts',(17.5098539640988,21.4609017047557,-13.1032927225808));
#47803=CARTESIAN_POINT('Ctrl Pts',(17.5841668423744,21.4997817138926,-13.1074773569739));
#47804=CARTESIAN_POINT('Ctrl Pts',(17.660324806961,21.5349667768392,-13.1116619913669));
#47805=CARTESIAN_POINT('Ctrl Pts',(17.7363743701113,21.5701017582038,-13.1158406694508));
#47806=CARTESIAN_POINT('Ctrl Pts',(17.8142633889641,21.6015520487103,-13.1200193475348));
#47807=CARTESIAN_POINT('Ctrl Pts',(17.8935998508933,21.629124808479,-13.1241980256187));
#47808=CARTESIAN_POINT('Ctrl Pts',(17.9743583618844,21.6571917901503,-13.1284516035042));
#47809=CARTESIAN_POINT('Ctrl Pts',(18.0566163014189,21.6812406201864,-13.1327051813896));
#47810=CARTESIAN_POINT('Ctrl Pts',(18.1399366350501,21.701118213745,-13.136958759275));
#47811=CARTESIAN_POINT('Ctrl Pts',(18.2216416414276,21.7206104413645,-13.141129873253));
#47812=CARTESIAN_POINT('Ctrl Pts',(18.3043677482543,21.7360916126581,-13.1453009872309));
#47813=CARTESIAN_POINT('Ctrl Pts',(18.3876870934184,21.7474674984582,-13.1494721012089));
#47814=CARTESIAN_POINT('Ctrl Pts',(18.4709784799716,21.75883956697,-13.1536418155293));
#47815=CARTESIAN_POINT('Ctrl Pts',(18.5548622540875,21.76610902368,-13.1578115298496));
#47816=CARTESIAN_POINT('Ctrl Pts',(18.6389020976073,21.7692330599381,-13.16198124417));
#47817=CARTESIAN_POINT('Ctrl Pts',(18.7229389506288,21.7723569850297,-13.1661508101141));
#47818=CARTESIAN_POINT('Ctrl Pts',(18.8071314022652,21.7713357667235,-13.1703203760581));
#47819=CARTESIAN_POINT('Ctrl Pts',(18.8910411442612,21.7661786784898,-13.1744899420021));
#47820=CARTESIAN_POINT('Ctrl Pts',(18.9779010492718,21.7608402733959,-13.1788061047411));
#47821=CARTESIAN_POINT('Ctrl Pts',(19.0644574681807,21.7510697851064,-13.18312226748));
#47822=CARTESIAN_POINT('Ctrl Pts',(19.1502297723789,21.7369360198915,-13.1874384302189));
#47823=CARTESIAN_POINT('Ctrl Pts',(19.2332080527895,21.7232626605919,-13.1916139944106));
#47824=CARTESIAN_POINT('Ctrl Pts',(19.3154520685911,21.7055060719794,-13.1957895586023));
#47825=CARTESIAN_POINT('Ctrl Pts',(19.3965387044154,21.6837803107335,-13.1999651227939));
#47826=CARTESIAN_POINT('Ctrl Pts',(19.4817208334499,21.6609572329353,-13.2043515848065));
#47827=CARTESIAN_POINT('Ctrl Pts',(19.5656250358875,21.6337536591884,-13.208738046819));
#47828=CARTESIAN_POINT('Ctrl Pts',(19.6477828618951,21.6023596302745,-13.2131245088315));
#47829=CARTESIAN_POINT('Ctrl Pts',(19.7299406879028,21.5709656013606,-13.2175109708441));
#47830=CARTESIAN_POINT('Ctrl Pts',(19.8103516376766,21.5353814216376,-13.2218974328566));
#47831=CARTESIAN_POINT('Ctrl Pts',(19.8885775886019,21.4958524223455,-13.2262838948691));
#47832=CARTESIAN_POINT('Ctrl Pts',(19.9631842212833,21.4581523305529,-13.2304674063033));
#47833=CARTESIAN_POINT('Ctrl Pts',(20.0360812001486,21.4167240952575,-13.2346509177374));
#47834=CARTESIAN_POINT('Ctrl Pts',(20.1068712604686,21.3717462836204,-13.2388344291715));
#47835=CARTESIAN_POINT('Ctrl Pts',(20.1709100371252,21.3310580285051,-13.2426189570156));
#47836=CARTESIAN_POINT('Ctrl Pts',(20.2332245698872,21.2874656707164,-13.2464034848598));
#47837=CARTESIAN_POINT('Ctrl Pts',(20.2935358855687,21.2411349269503,-13.2501880127039));
#47838=CARTESIAN_POINT('Ctrl Pts',(20.2954167287344,21.2436206075649,-12.4500366863435));
#47839=CARTESIAN_POINT('Ctrl Pts',(20.3656979514168,21.1904720313874,-12.4544341424892));
#47840=CARTESIAN_POINT('Ctrl Pts',(21.0821531671319,20.5851355586758,-12.5012235341954));
#47841=CARTESIAN_POINT('Ctrl Pts',(21.7088252035205,18.6509044816894,-12.590404861462));
#47842=CARTESIAN_POINT('Ctrl Pts',(19.8732647667815,16.4064736991244,-12.7175806681434));
#47843=CARTESIAN_POINT('Ctrl Pts',(17.0319370398065,16.7305239353302,-12.8430154491721));
#47844=CARTESIAN_POINT('Ctrl Pts',(16.1727139355615,18.3978728515243,-12.9260582946402));
#47845=CARTESIAN_POINT('Ctrl Pts',(16.1699654719056,19.2116308397489,-12.9667092045479));
#47846=CARTESIAN_POINT('Origin',(18.734,19.211,1.76670989022852));
#47847=CARTESIAN_POINT('',(20.2935358855687,21.2411349269503,-11.650072531177));
#47848=CARTESIAN_POINT('',(20.2935358855687,21.2411349269503,-11.7167617888358));
#47849=CARTESIAN_POINT('',(20.2935358855687,21.2411349269503,1.76670989022852));
#47850=CARTESIAN_POINT('',(16.1740010233873,19.2087109517327,-12.2332901098107));
#47851=CARTESIAN_POINT('Ctrl Pts',(20.2935358855687,21.2411349269503,-11.7167617888358));
#47852=CARTESIAN_POINT('Ctrl Pts',(20.3600167937585,21.1900647440522,-11.7209383136263));
#47853=CARTESIAN_POINT('Ctrl Pts',(20.4240745352904,21.135657894152,-11.7251148384167));
#47854=CARTESIAN_POINT('Ctrl Pts',(20.4853583496099,21.0781753884549,-11.7292913632071));
#47855=CARTESIAN_POINT('Ctrl Pts',(20.5465832892312,21.0207481055799,-11.7334638756552));
#47856=CARTESIAN_POINT('Ctrl Pts',(20.6050392636091,20.9602513525623,-11.7376363881034));
#47857=CARTESIAN_POINT('Ctrl Pts',(20.6604085763013,20.8969863573448,-11.7418089005516));
#47858=CARTESIAN_POINT('Ctrl Pts',(20.7157495989849,20.8337536863006,-11.7459792811255));
#47859=CARTESIAN_POINT('Ctrl Pts',(20.7680067888956,20.7677559268922,-11.7501496616994));
#47860=CARTESIAN_POINT('Ctrl Pts',(20.8169001522236,20.6993302576602,-11.7543200422733));
#47861=CARTESIAN_POINT('Ctrl Pts',(20.865783201272,20.6309190231374,-11.7584895430863));
#47862=CARTESIAN_POINT('Ctrl Pts',(20.9113035661553,20.5600812704941,-11.7626590438993));
#47863=CARTESIAN_POINT('Ctrl Pts',(20.9532231556077,20.4871851690152,-11.7668285447122));
#47864=CARTESIAN_POINT('Ctrl Pts',(20.9951464766831,20.4142825784279,-11.7709984166883));
#47865=CARTESIAN_POINT('Ctrl Pts',(21.0334681576709,20.3393216746274,-11.7751682886644));
#47866=CARTESIAN_POINT('Ctrl Pts',(21.0679955410099,20.2626961607546,-11.7793381606404));
#47867=CARTESIAN_POINT('Ctrl Pts',(21.1025593312112,20.1859898503005,-11.7835124294732));
#47868=CARTESIAN_POINT('Ctrl Pts',(21.1333206459673,20.1076158454035,-11.7876866983059));
#47869=CARTESIAN_POINT('Ctrl Pts',(21.1601347931878,20.0279883507638,-11.7918609671386));
#47870=CARTESIAN_POINT('Ctrl Pts',(21.1869637575432,19.9483168550479,-11.7960375426158));
#47871=CARTESIAN_POINT('Ctrl Pts',(21.2098410861947,19.8673909332363,-11.800214118093));
#47872=CARTESIAN_POINT('Ctrl Pts',(21.2286725239124,19.7856381456505,-11.8043906935702));
#47873=CARTESIAN_POINT('Ctrl Pts',(21.24753646193,19.7037442647422,-11.8085744772042));
#47874=CARTESIAN_POINT('Ctrl Pts',(21.2623404822881,19.621021121095,-11.8127582608381));
#47875=CARTESIAN_POINT('Ctrl Pts',(21.2730418536683,19.5379043672401,-11.8169420444721));
#47876=CARTESIAN_POINT('Ctrl Pts',(21.280709708626,19.4783487093277,-11.8199398514765));
#47877=CARTESIAN_POINT('Ctrl Pts',(21.2862722939427,19.4185911058323,-11.8229376584808));
#47878=CARTESIAN_POINT('Ctrl Pts',(21.2897303495757,19.3587916785811,-11.8259354654852));
#47879=CARTESIAN_POINT('Ctrl Pts',(21.2945574443532,19.2753177459375,-11.8301200998782));
#47880=CARTESIAN_POINT('Ctrl Pts',(21.295299648515,19.1914517330296,-11.8343047342713));
#47881=CARTESIAN_POINT('Ctrl Pts',(21.2919120526423,19.1076272233756,-11.8384893686643));
#47882=CARTESIAN_POINT('Ctrl Pts',(21.2885292785931,19.0239220275358,-11.8426680467483));
#47883=CARTESIAN_POINT('Ctrl Pts',(21.2810283989992,18.940258673335,-11.8468467248322));
#47884=CARTESIAN_POINT('Ctrl Pts',(21.2694164102341,18.8570739812961,-11.8510254029161));
#47885=CARTESIAN_POINT('Ctrl Pts',(21.2575962849158,18.772398263436,-11.8552789808016));
#47886=CARTESIAN_POINT('Ctrl Pts',(21.2415161896732,18.6882190178967,-11.859532558687));
#47887=CARTESIAN_POINT('Ctrl Pts',(21.221239025086,18.604995023049,-11.8637861365725));
#47888=CARTESIAN_POINT('Ctrl Pts',(21.2013549729019,18.5233844877397,-11.8679572505504));
#47889=CARTESIAN_POINT('Ctrl Pts',(21.1774352498115,18.4426929623941,-11.8721283645284));
#47890=CARTESIAN_POINT('Ctrl Pts',(21.1495909652084,18.3633442392081,-11.8762994785063));
#47891=CARTESIAN_POINT('Ctrl Pts',(21.1217560240238,18.2840221422525,-11.8804691928267));
#47892=CARTESIAN_POINT('Ctrl Pts',(21.0899992889567,18.2060423862984,-11.8846389071471));
#47893=CARTESIAN_POINT('Ctrl Pts',(21.0544814935988,18.1298128571493,-11.8888086214674));
#47894=CARTESIAN_POINT('Ctrl Pts',(21.0189649621164,18.0535860405741,-11.8929781874115));
#47895=CARTESIAN_POINT('Ctrl Pts',(20.9796878315031,17.9791097436055,-11.8971477533555));
#47896=CARTESIAN_POINT('Ctrl Pts',(20.9368581017986,17.9067698886545,-11.9013173192996));
#47897=CARTESIAN_POINT('Ctrl Pts',(20.8925225316338,17.8318866536443,-11.9056334820385));
#47898=CARTESIAN_POINT('Ctrl Pts',(20.8443801641988,17.7592933443553,-11.9099496447774));
#47899=CARTESIAN_POINT('Ctrl Pts',(20.7927112772811,17.6893864233007,-11.9142658075163));
#47900=CARTESIAN_POINT('Ctrl Pts',(20.7427254989202,17.6217567128466,-11.918441371708));
#47901=CARTESIAN_POINT('Ctrl Pts',(20.6894397604074,17.5566413947911,-11.9226169358997));
#47902=CARTESIAN_POINT('Ctrl Pts',(20.6331484080961,17.4943651162737,-11.9267925000914));
#47903=CARTESIAN_POINT('Ctrl Pts',(20.5740139133994,17.4289434109761,-11.9311789621039));
#47904=CARTESIAN_POINT('Ctrl Pts',(20.5115626117394,17.3666554945532,-11.9355654241165));
#47905=CARTESIAN_POINT('Ctrl Pts',(20.4461771444977,17.3078317400031,-11.939951886129));
#47906=CARTESIAN_POINT('Ctrl Pts',(20.3807916772559,17.2490079854529,-11.9443383481416));
#47907=CARTESIAN_POINT('Ctrl Pts',(20.3124725431188,17.1936486989611,-11.9487248101541));
#47908=CARTESIAN_POINT('Ctrl Pts',(20.2416377781113,17.1420320616279,-11.9531112721667));
#47909=CARTESIAN_POINT('Ctrl Pts',(20.1740622256442,17.0927903822927,-11.9572959065597));
#47910=CARTESIAN_POINT('Ctrl Pts',(20.1039459219087,17.0467712239067,-11.9614805409528));
#47911=CARTESIAN_POINT('Ctrl Pts',(20.0316291334109,17.0042470387188,-11.9656651753458));
#47912=CARTESIAN_POINT('Ctrl Pts',(19.9594152789105,16.9617833814451,-11.9698438534298));
#47913=CARTESIAN_POINT('Ctrl Pts',(19.8850075541817,16.9228050473158,-11.9740225315137));
#47914=CARTESIAN_POINT('Ctrl Pts',(19.8087770431601,16.887542596152,-11.9782012095977));
#47915=CARTESIAN_POINT('Ctrl Pts',(19.7311801550143,16.8516480908937,-11.9824547874831));
#47916=CARTESIAN_POINT('Ctrl Pts',(19.6516948805984,16.8196042772378,-11.9867083653685));
#47917=CARTESIAN_POINT('Ctrl Pts',(19.57074102681,16.7916065937816,-11.990961943254));
#47918=CARTESIAN_POINT('Ctrl Pts',(19.4913566214457,16.7641517000523,-11.9951330572319));
#47919=CARTESIAN_POINT('Ctrl Pts',(19.4105605259053,16.7405876095593,-11.9993041712099));
#47920=CARTESIAN_POINT('Ctrl Pts',(19.3287692237664,16.721050287564,-12.0034752851878));
#47921=CARTESIAN_POINT('Ctrl Pts',(19.2470053674889,16.7015195215057,-12.0076449995082));
#47922=CARTESIAN_POINT('Ctrl Pts',(19.1642474149177,16.68601294719,-12.0118147138286));
#47923=CARTESIAN_POINT('Ctrl Pts',(19.0809253355089,16.6746161939521,-12.015984428149));
#47924=CARTESIAN_POINT('Ctrl Pts',(18.9976062210572,16.6632198462596,-12.020153994093));
#47925=CARTESIAN_POINT('Ctrl Pts',(18.9137234755848,16.6559330903703,-12.024323560037));
#47926=CARTESIAN_POINT('Ctrl Pts',(18.8297141852422,16.6527899236491,-12.0284931259811));
#47927=CARTESIAN_POINT('Ctrl Pts',(18.7427512318879,16.6495362470634,-12.03280928872));
#47928=CARTESIAN_POINT('Ctrl Pts',(18.6556531965159,16.6507229779044,-12.0371254514589));
#47929=CARTESIAN_POINT('Ctrl Pts',(18.5689051504086,16.6563290445464,-12.0414416141978));
#47930=CARTESIAN_POINT('Ctrl Pts',(18.4849829127789,16.6617524941571,-12.0456171783895));
#47931=CARTESIAN_POINT('Ctrl Pts',(18.4013886754037,16.6713116809417,-12.0497927425812));
#47932=CARTESIAN_POINT('Ctrl Pts',(18.3185547392491,16.6849348315375,-12.0539683067729));
#47933=CARTESIAN_POINT('Ctrl Pts',(18.2315370578984,16.6992460550839,-12.0583547687854));
#47934=CARTESIAN_POINT('Ctrl Pts',(18.1453590723574,16.7180424488713,-12.062741230798));
#47935=CARTESIAN_POINT('Ctrl Pts',(18.0605056905574,16.7411810966898,-12.0671276928105));
#47936=CARTESIAN_POINT('Ctrl Pts',(17.9756523087575,16.7643197445083,-12.071514154823));
#47937=CARTESIAN_POINT('Ctrl Pts',(17.8921240580815,16.7918003927741,-12.0759006168356));
#47938=CARTESIAN_POINT('Ctrl Pts',(17.8103811197834,16.8234221134992,-12.0802870788481));
#47939=CARTESIAN_POINT('Ctrl Pts',(17.7323992952485,16.8535888719792,-12.0844717132412));
#47940=CARTESIAN_POINT('Ctrl Pts',(17.6557518403844,16.8876362896632,-12.0886563476342));
#47941=CARTESIAN_POINT('Ctrl Pts',(17.5808520242221,16.9254257295027,-12.0928409820273));
#47942=CARTESIAN_POINT('Ctrl Pts',(17.5060588186774,16.963161380752,-12.0970196601112));
#47943=CARTESIAN_POINT('Ctrl Pts',(17.4330087179883,17.0046282689895,-12.1011983381951));
#47944=CARTESIAN_POINT('Ctrl Pts',(17.3620964471734,17.0496391690091,-12.1053770162791));
#47945=CARTESIAN_POINT('Ctrl Pts',(17.2899131248678,17.0954568570628,-12.1096305941645));
#47946=CARTESIAN_POINT('Ctrl Pts',(17.2199454771428,17.1449466854561,-12.11388417205));
#47947=CARTESIAN_POINT('Ctrl Pts',(17.1525850704413,17.1978614502303,-12.1181377499354));
#47948=CARTESIAN_POINT('Ctrl Pts',(17.0865305766667,17.2497503590347,-12.1223088639134));
#47949=CARTESIAN_POINT('Ctrl Pts',(17.0229835115634,17.3049322938693,-12.1264799778913));
#47950=CARTESIAN_POINT('Ctrl Pts',(16.9622836350606,17.3631306533724,-12.1306510918693));
#47951=CARTESIAN_POINT('Ctrl Pts',(16.9016041269875,17.421309483854,-12.1348208061896));
#47952=CARTESIAN_POINT('Ctrl Pts',(16.8437702418585,17.4825024106647,-12.13899052051));
#47953=CARTESIAN_POINT('Ctrl Pts',(16.789086714705,17.5463942470714,-12.1431602348304));
#47954=CARTESIAN_POINT('Ctrl Pts',(16.734405133426,17.6102838099324,-12.1473298007744));
#47955=CARTESIAN_POINT('Ctrl Pts',(16.6828739857151,17.6768717413838,-12.1514993667185));
#47956=CARTESIAN_POINT('Ctrl Pts',(16.6347584444193,17.7458089232721,-12.1556689326625));
#47957=CARTESIAN_POINT('Ctrl Pts',(16.5849512200484,17.8171698514323,-12.1599850954014));
#47958=CARTESIAN_POINT('Ctrl Pts',(16.5388045582795,17.8910478705134,-12.1643012581403));
#47959=CARTESIAN_POINT('Ctrl Pts',(16.496563301095,17.9670237066595,-12.1686174208793));
#47960=CARTESIAN_POINT('Ctrl Pts',(16.4556980484203,18.0405246379344,-12.1727929850709));
#47961=CARTESIAN_POINT('Ctrl Pts',(16.4184878365309,18.1159883689942,-12.1769685492626));
#47962=CARTESIAN_POINT('Ctrl Pts',(16.3851063117011,18.1930125535796,-12.1811441134543));
#47963=CARTESIAN_POINT('Ctrl Pts',(16.3500387654091,18.2739270466208,-12.1855305754669));
#47964=CARTESIAN_POINT('Ctrl Pts',(16.3191970489119,18.3565632259542,-12.1899170374794));
#47965=CARTESIAN_POINT('Ctrl Pts',(16.2927234637602,18.4404360029142,-12.1943034994919));
#47966=CARTESIAN_POINT('Ctrl Pts',(16.2662498786085,18.5243087798742,-12.1986899615045));
#47967=CARTESIAN_POINT('Ctrl Pts',(16.2441444970407,18.6094175737551,-12.203076423517));
#47968=CARTESIAN_POINT('Ctrl Pts',(16.2264874578015,18.6952666864385,-12.2074628855296));
#47969=CARTESIAN_POINT('Ctrl Pts',(16.2025156137663,18.811818590295,-12.2134181072293));
#47970=CARTESIAN_POINT('Ctrl Pts',(16.1866633864877,18.9300931627176,-12.219373328929));
#47971=CARTESIAN_POINT('Ctrl Pts',(16.1791211348988,19.0491544419537,-12.2253285506288));
#47972=CARTESIAN_POINT('Ctrl Pts',(16.1757600463661,19.10221227165,-12.2279824036764));
#47973=CARTESIAN_POINT('Ctrl Pts',(16.1740486686438,19.1554260264049,-12.2306362567239));
#47974=CARTESIAN_POINT('Ctrl Pts',(16.174001023388,19.2087109509454,-12.2332901097715));
#47975=CARTESIAN_POINT('Ctrl Pts',(16.1740010233873,19.2087109517327,-12.2332901098107));
#47976=CARTESIAN_POINT('Ctrl Pts',(16.1739252094451,19.293498859929,-12.2375129674107));
#47977=CARTESIAN_POINT('Ctrl Pts',(16.1780663695147,19.3784221563148,-12.2417358250107));
#47978=CARTESIAN_POINT('Ctrl Pts',(16.1864353355331,19.4630203967139,-12.2459586826108));
#47979=CARTESIAN_POINT('Ctrl Pts',(16.1945865434513,19.5454174151127,-12.2500716626647));
#47980=CARTESIAN_POINT('Ctrl Pts',(16.2067481850334,19.6275055813485,-12.2541846427187));
#47981=CARTESIAN_POINT('Ctrl Pts',(16.2228775801224,19.7088596111236,-12.2582976227727));
#47982=CARTESIAN_POINT('Ctrl Pts',(16.2389992540558,19.7901746966527,-12.2624086339395));
#47983=CARTESIAN_POINT('Ctrl Pts',(16.25908482094,19.8707558783837,-12.2665196451063));
#47984=CARTESIAN_POINT('Ctrl Pts',(16.2830401055299,19.9501857653521,-12.2706306562731));
#47985=CARTESIAN_POINT('Ctrl Pts',(16.3069915898918,20.0296030516901,-12.2747410152757));
#47986=CARTESIAN_POINT('Ctrl Pts',(16.3348114354692,20.1078689519365,-12.2788513742782));
#47987=CARTESIAN_POINT('Ctrl Pts',(16.366355393672,20.1845805144548,-12.2829617332808));
#47988=CARTESIAN_POINT('Ctrl Pts',(16.3994039228381,20.264951034063,-12.2872681465249));
#47989=CARTESIAN_POINT('Ctrl Pts',(16.4365404963283,20.3436147061446,-12.2915745597691));
#47990=CARTESIAN_POINT('Ctrl Pts',(16.4775431085385,20.4201328698599,-12.2958809730133));
#47991=CARTESIAN_POINT('Ctrl Pts',(16.5167281737211,20.4932591677035,-12.2999964933322));
#47992=CARTESIAN_POINT('Ctrl Pts',(16.5594435017451,20.5644257408165,-12.304112013651));
#47993=CARTESIAN_POINT('Ctrl Pts',(16.6054498638678,20.6332778624347,-12.3082275339699));
#47994=CARTESIAN_POINT('Ctrl Pts',(16.6514869443887,20.7021759565399,-12.3123458022172));
#47995=CARTESIAN_POINT('Ctrl Pts',(16.7008191449123,20.768756147345,-12.3164640704645));
#47996=CARTESIAN_POINT('Ctrl Pts',(16.7531665958489,20.8326963417974,-12.3205823387118));
#47997=CARTESIAN_POINT('Ctrl Pts',(16.8055945346489,20.8967348487664,-12.3247069390843));
#47998=CARTESIAN_POINT('Ctrl Pts',(16.8610466479906,20.9581249187389,-12.3288315394568));
#47999=CARTESIAN_POINT('Ctrl Pts',(16.9192065009781,21.0165815007659,-12.3329561398293));
#48000=CARTESIAN_POINT('Ctrl Pts',(16.9271149034352,21.0245302515482,-12.3335169906232));
#48001=CARTESIAN_POINT('Ctrl Pts',(16.93507332294,21.0324248251516,-12.3340778414171));
#48002=CARTESIAN_POINT('Ctrl Pts',(16.9430809195058,21.040264564551,-12.334638692211));
#48003=CARTESIAN_POINT('Ctrl Pts',(17.0028274053093,21.0987586301397,-12.338823326604));
#48004=CARTESIAN_POINT('Ctrl Pts',(17.0655538444182,21.1544313597729,-12.3430079609971));
#48005=CARTESIAN_POINT('Ctrl Pts',(17.1309629349571,21.2069639696394,-12.3471925953901));
#48006=CARTESIAN_POINT('Ctrl Pts',(17.1962789237517,21.259421805838,-12.3513712734741));
#48007=CARTESIAN_POINT('Ctrl Pts',(17.2642696237805,21.3087481146435,-12.355549951558));
#48008=CARTESIAN_POINT('Ctrl Pts',(17.3346011829193,21.3546611091199,-12.3597286296419));
#48009=CARTESIAN_POINT('Ctrl Pts',(17.4061933847094,21.4013970610253,-12.3639822075274));
#48010=CARTESIAN_POINT('Ctrl Pts',(17.4802108463241,21.4445957903897,-12.3682357854128));
#48011=CARTESIAN_POINT('Ctrl Pts',(17.5562664269212,21.484003218397,-12.3724893632982));
#48012=CARTESIAN_POINT('Ctrl Pts',(17.6308475216781,21.522646656515,-12.3766604772762));
#48013=CARTESIAN_POINT('Ctrl Pts',(17.7073879875327,21.5576442636058,-12.3808315912541));
#48014=CARTESIAN_POINT('Ctrl Pts',(17.7854953736982,21.5888012898231,-12.3850027052321));
#48015=CARTESIAN_POINT('Ctrl Pts',(17.863576550176,21.6199478609992,-12.3891724195525));
#48016=CARTESIAN_POINT('Ctrl Pts',(17.9432231757909,21.6472562404631,-12.3933421338728));
#48017=CARTESIAN_POINT('Ctrl Pts',(18.0240221782528,21.6705795357392,-12.3975118481932));
#48018=CARTESIAN_POINT('Ctrl Pts',(18.1048183055395,21.6939020010724,-12.4016814141373));
#48019=CARTESIAN_POINT('Ctrl Pts',(18.186766285918,21.713239537401,-12.4058509800813));
#48020=CARTESIAN_POINT('Ctrl Pts',(18.2694385404879,21.7284953128727,-12.4100205460253));
#48021=CARTESIAN_POINT('Ctrl Pts',(18.3550174495411,21.7442874625899,-12.4143367087643));
#48022=CARTESIAN_POINT('Ctrl Pts',(18.4413719926986,21.7557053858609,-12.4186528715032));
#48023=CARTESIAN_POINT('Ctrl Pts',(18.5280191484746,21.762699803818,-12.4229690342421));
#48024=CARTESIAN_POINT('Ctrl Pts',(18.6118437822649,21.7694663793459,-12.4271445984338));
#48025=CARTESIAN_POINT('Ctrl Pts',(18.6959417854331,21.7720932477196,-12.4313201626255));
#48026=CARTESIAN_POINT('Ctrl Pts',(18.7798750222012,21.7705889283903,-12.4354957268171));
#48027=CARTESIAN_POINT('Ctrl Pts',(18.8680475272262,21.7690086294678,-12.4398821888297));
#48028=CARTESIAN_POINT('Ctrl Pts',(18.9560376012523,21.7628688832023,-12.4442686508422));
#48029=CARTESIAN_POINT('Ctrl Pts',(19.0433447687653,21.7522409988109,-12.4486551128548));
#48030=CARTESIAN_POINT('Ctrl Pts',(19.1306519362783,21.7416131144196,-12.4530415748673));
#48031=CARTESIAN_POINT('Ctrl Pts',(19.2172756387742,21.7264972665759,-12.4574280368799));
#48032=CARTESIAN_POINT('Ctrl Pts',(19.3027314805894,21.7070257416514,-12.4618144988924));
#48033=CARTESIAN_POINT('Ctrl Pts',(19.3842631981423,21.6884483473301,-12.4659995349797));
#48034=CARTESIAN_POINT('Ctrl Pts',(19.4650354649563,21.6658373731213,-12.4701845710669));
#48035=CARTESIAN_POINT('Ctrl Pts',(19.5446191872091,21.6392702760048,-12.4743696071542));
#48036=CARTESIAN_POINT('Ctrl Pts',(19.6240693838798,21.6127477531682,-12.4785476215872));
#48037=CARTESIAN_POINT('Ctrl Pts',(19.7023345681446,21.5822824489793,-12.4827256360202));
#48038=CARTESIAN_POINT('Ctrl Pts',(19.7789972930808,21.5480024941052,-12.4869036504532));
#48039=CARTESIAN_POINT('Ctrl Pts',(19.8555857432778,21.5137557513914,-12.4910776170138));
#48040=CARTESIAN_POINT('Ctrl Pts',(19.9305743987691,21.4757018818008,-12.4952515835744));
#48041=CARTESIAN_POINT('Ctrl Pts',(20.003563194091,21.4340180602527,-12.4994255501349));
#48042=CARTESIAN_POINT('Ctrl Pts',(20.0764986900058,21.392364677938,-12.5035964686942));
#48043=CARTESIAN_POINT('Ctrl Pts',(20.1474368294337,21.3470868385682,-12.5077673872535));
#48044=CARTESIAN_POINT('Ctrl Pts',(20.2160009920406,21.2984082158483,-12.5119383058127));
#48045=CARTESIAN_POINT('Ctrl Pts',(20.2421989287405,21.2798084192757,-12.5135319876465));
#48046=CARTESIAN_POINT('Ctrl Pts',(20.2680505424068,21.2607125947641,-12.5151256694803));
#48047=CARTESIAN_POINT('Ctrl Pts',(20.2935358855687,21.2411349269503,-12.5167193513141));
#48048=CARTESIAN_POINT('',(16.1740007840082,19.2130035272629,-12.1667098902285));
#48049=CARTESIAN_POINT('Ctrl Pts',(16.1763509819005,19.2130199893541,-12.1667107986141));
#48050=CARTESIAN_POINT('Ctrl Pts',(16.174290235218,19.4962014494758,-12.1807663462153));
#48051=CARTESIAN_POINT('Ctrl Pts',(16.3483939114844,20.6310006362221,-12.237213829377));
#48052=CARTESIAN_POINT('Ctrl Pts',(17.9381456425209,22.083154657165,-12.3316557919534));
#48053=CARTESIAN_POINT('Ctrl Pts',(19.6881796398412,21.7028298450405,-12.4120422069287));
#48054=CARTESIAN_POINT('Ctrl Pts',(20.2954167287344,21.2436206075649,-12.4500366863435));
#48055=CARTESIAN_POINT('Ctrl Pts',(20.2935358855687,21.2411349269503,-11.650072531177));
#48056=CARTESIAN_POINT('Ctrl Pts',(20.3602862218061,21.1898577712529,-11.6542476714699));
#48057=CARTESIAN_POINT('Ctrl Pts',(20.4244786660862,21.1353052511714,-11.6584228117628));
#48058=CARTESIAN_POINT('Ctrl Pts',(20.485787760444,21.0777725202494,-11.6625979520557));
#48059=CARTESIAN_POINT('Ctrl Pts',(20.5471067961931,21.0202304602811,-11.6667737693559));
#48060=CARTESIAN_POINT('Ctrl Pts',(20.6055412401485,20.9597075680707,-11.6709495866561));
#48061=CARTESIAN_POINT('Ctrl Pts',(20.6608038249164,20.8965346393022,-11.6751254039563));
#48062=CARTESIAN_POINT('Ctrl Pts',(20.7161667197055,20.8332470420314,-11.6793088010019));
#48063=CARTESIAN_POINT('Ctrl Pts',(20.768345963538,20.7673001572432,-11.6834921980475));
#48064=CARTESIAN_POINT('Ctrl Pts',(20.8170955352535,20.6990567835292,-11.687675595093));
#48065=CARTESIAN_POINT('Ctrl Pts',(20.8656447840932,20.6310938370762,-11.691841801626));
#48066=CARTESIAN_POINT('Ctrl Pts',(20.9107923286134,20.560853665295,-11.696008008159));
#48067=CARTESIAN_POINT('Ctrl Pts',(20.9523407266398,20.4887184433713,-11.700174214692));
#48068=CARTESIAN_POINT('Ctrl Pts',(20.9940729004966,20.4162641547461,-11.704358849085));
#48069=CARTESIAN_POINT('Ctrl Pts',(21.0323293070735,20.3416283299438,-11.7085434834781));
#48070=CARTESIAN_POINT('Ctrl Pts',(21.06687544764,20.265178422184,-11.7127281178711));
#48071=CARTESIAN_POINT('Ctrl Pts',(21.1013724160514,20.1888373314053,-11.7169067959551));
#48072=CARTESIAN_POINT('Ctrl Pts',(21.1321694205716,20.11068770221,-11.721085474039));
#48073=CARTESIAN_POINT('Ctrl Pts',(21.159076910497,20.0311231481761,-11.725264152123));
#48074=CARTESIAN_POINT('Ctrl Pts',(21.1864666978413,19.9501324566932,-11.7295177300084));
#48075=CARTESIAN_POINT('Ctrl Pts',(21.2098259193361,19.8676760341796,-11.7337713078938));
#48076=CARTESIAN_POINT('Ctrl Pts',(21.2290051549002,19.7841921815775,-11.7380248857793));
#48077=CARTESIAN_POINT('Ctrl Pts',(21.2478125635577,19.7023268263635,-11.7421959997572));
#48078=CARTESIAN_POINT('Ctrl Pts',(21.2626005065823,19.6194739920339,-11.7463671137352));
#48079=CARTESIAN_POINT('Ctrl Pts',(21.2732783407021,19.5360623147049,-11.7505382277131));
#48080=CARTESIAN_POINT('Ctrl Pts',(21.2839525917715,19.4526786269698,-11.7547079420335));
#48081=CARTESIAN_POINT('Ctrl Pts',(21.2905194146576,19.3687369245927,-11.7588776563539));
#48082=CARTESIAN_POINT('Ctrl Pts',(21.2929396556081,19.2846738688838,-11.7630473706742));
#48083=CARTESIAN_POINT('Ctrl Pts',(21.295359810436,19.2006138044992,-11.7672169366183));
#48084=CARTESIAN_POINT('Ctrl Pts',(21.2936336643145,19.1164328552356,-11.7713865025623));
#48085=CARTESIAN_POINT('Ctrl Pts',(21.2877741604491,19.0325692363337,-11.7755560685064));
#48086=CARTESIAN_POINT('Ctrl Pts',(21.2817086436563,18.945757076048,-11.7798722312453));
#48087=CARTESIAN_POINT('Ctrl Pts',(21.2712137402019,18.859285502122,-11.7841883939842));
#48088=CARTESIAN_POINT('Ctrl Pts',(21.2563622783628,18.7736345501841,-11.7885045567231));
#48089=CARTESIAN_POINT('Ctrl Pts',(21.241994601331,18.6907736689967,-11.7926801209148));
#48090=CARTESIAN_POINT('Ctrl Pts',(21.2235499863026,18.6086812165374,-11.7968556851065));
#48091=CARTESIAN_POINT('Ctrl Pts',(21.2011460288054,18.5277793383177,-11.8010312492982));
#48092=CARTESIAN_POINT('Ctrl Pts',(21.1776105006754,18.442791298555,-11.8054177113107));
#48093=CARTESIAN_POINT('Ctrl Pts',(21.1497053305466,18.3591178195345,-11.8098041733232));
#48094=CARTESIAN_POINT('Ctrl Pts',(21.1176244749813,18.27722574341,-11.8141906353358));
#48095=CARTESIAN_POINT('Ctrl Pts',(21.085543619416,18.1953336672855,-11.8185770973483));
#48096=CARTESIAN_POINT('Ctrl Pts',(21.0492873869465,18.115223491295,-11.8229635593609));
#48097=CARTESIAN_POINT('Ctrl Pts',(21.0091047687183,18.0373312684769,-11.8273500213734));
#48098=CARTESIAN_POINT('Ctrl Pts',(20.9707710123198,17.9630229822945,-11.8315346557664));
#48099=CARTESIAN_POINT('Ctrl Pts',(20.9287215623263,17.8904564421858,-11.8357192901595));
#48100=CARTESIAN_POINT('Ctrl Pts',(20.8831384590298,17.8200277199315,-11.8399039245525));
#48101=CARTESIAN_POINT('Ctrl Pts',(20.8376202376387,17.7496992442458,-11.8440826026365));
#48102=CARTESIAN_POINT('Ctrl Pts',(20.7885786013676,17.6815029251172,-11.8482612807204));
#48103=CARTESIAN_POINT('Ctrl Pts',(20.7362419167444,17.615811200255,-11.8524399588044));
#48104=CARTESIAN_POINT('Ctrl Pts',(20.682967134663,17.5489419984366,-11.8566935366898));
#48105=CARTESIAN_POINT('Ctrl Pts',(20.6262782358934,17.4846684922396,-11.8609471145753));
#48106=CARTESIAN_POINT('Ctrl Pts',(20.566462883909,17.423353564293,-11.8652006924607));
#48107=CARTESIAN_POINT('Ctrl Pts',(20.5078071692429,17.3632273458709,-11.8693718064386));
#48108=CARTESIAN_POINT('Ctrl Pts',(20.4461454804008,17.3059463582357,-11.8735429204166));
#48109=CARTESIAN_POINT('Ctrl Pts',(20.3817891690391,17.2518188306343,-11.8777140343945));
#48110=CARTESIAN_POINT('Ctrl Pts',(20.3174544530593,17.1977094660475,-11.8818837487149));
#48111=CARTESIAN_POINT('Ctrl Pts',(20.2504272621012,17.1467517558061,-11.8860534630353));
#48112=CARTESIAN_POINT('Ctrl Pts',(20.1810535660399,17.0992149785049,-11.8902231773557));
#48113=CARTESIAN_POINT('Ctrl Pts',(20.1116823385924,17.0516798927661,-11.8943927432997));
#48114=CARTESIAN_POINT('Ctrl Pts',(20.0399651520288,17.0075657572672,-11.8985623092438));
#48115=CARTESIAN_POINT('Ctrl Pts',(19.9662774819293,16.967098886419,-11.9027318751878));
#48116=CARTESIAN_POINT('Ctrl Pts',(19.8899990442531,16.9252092503133,-11.9070480379267));
#48117=CARTESIAN_POINT('Ctrl Pts',(19.8116094428164,16.887228380361,-11.9113642006657));
#48118=CARTESIAN_POINT('Ctrl Pts',(19.7315517321804,16.8533548736877,-11.9156803634046));
#48119=CARTESIAN_POINT('Ctrl Pts',(19.6541018930477,16.8205847929315,-11.9198559275963));
#48120=CARTESIAN_POINT('Ctrl Pts',(19.5750914116565,16.791658707737,-11.9240314917879));
#48121=CARTESIAN_POINT('Ctrl Pts',(19.4949388978049,16.7667062382341,-11.9282070559796));
#48122=CARTESIAN_POINT('Ctrl Pts',(19.4107380710233,16.7404934788156,-11.9325935179922));
#48123=CARTESIAN_POINT('Ctrl Pts',(19.325277377455,16.7186664436044,-11.9369799800047));
#48124=CARTESIAN_POINT('Ctrl Pts',(19.2390543424806,16.7013147386293,-11.9413664420172));
#48125=CARTESIAN_POINT('Ctrl Pts',(19.1528313075062,16.6839630336542,-11.9457529040298));
#48126=CARTESIAN_POINT('Ctrl Pts',(19.0658465162266,16.6710866686339,-11.9501393660423));
#48127=CARTESIAN_POINT('Ctrl Pts',(18.9786013944249,16.662712308658,-11.9545258280548));
#48128=CARTESIAN_POINT('Ctrl Pts',(18.8953705500055,16.6547232653983,-11.9587104624479));
#48129=CARTESIAN_POINT('Ctrl Pts',(18.8115930039275,16.6508013065455,-11.9628950968409));
#48130=CARTESIAN_POINT('Ctrl Pts',(18.727700324836,16.6510077511655,-11.967079731234));
#48131=CARTESIAN_POINT('Ctrl Pts',(18.6439270565895,16.6512139019371,-11.9712584093179));
#48132=CARTESIAN_POINT('Ctrl Pts',(18.5600394369387,16.655536782935,-11.9754370874018));
#48133=CARTESIAN_POINT('Ctrl Pts',(18.4764742375278,16.6639859675174,-11.9796157654858));
#48134=CARTESIAN_POINT('Ctrl Pts',(18.3914111919746,16.6725865976612,-11.9838693433712));
#48135=CARTESIAN_POINT('Ctrl Pts',(18.3066827190517,16.6854629604527,-11.9881229212567));
#48136=CARTESIAN_POINT('Ctrl Pts',(18.2227496524051,16.702569597919,-11.9923764991421));
#48137=CARTESIAN_POINT('Ctrl Pts',(18.1404437920373,16.7193445898372,-11.9965476131201));
#48138=CARTESIAN_POINT('Ctrl Pts',(18.0589032436851,16.7401871997925,-12.000718727098));
#48139=CARTESIAN_POINT('Ctrl Pts',(17.9785557081131,16.7650024689597,-12.004889841076));
#48140=CARTESIAN_POINT('Ctrl Pts',(17.8982351339326,16.7898094111236,-12.0090595553964));
#48141=CARTESIAN_POINT('Ctrl Pts',(17.8191072166575,16.8185862293723,-12.0132292697167));
#48142=CARTESIAN_POINT('Ctrl Pts',(17.7415856439034,16.8511877731876,-12.0173989840371));
#48143=CARTESIAN_POINT('Ctrl Pts',(17.6640668296998,16.8837881569,-12.0215685499812));
#48144=CARTESIAN_POINT('Ctrl Pts',(17.5881546700958,16.9202128164542,-12.0257381159252));
#48145=CARTESIAN_POINT('Ctrl Pts',(17.5142426975062,16.9602685360059,-12.0299076818693));
#48146=CARTESIAN_POINT('Ctrl Pts',(17.4377320711406,17.0017325652429,-12.0342238446082));
#48147=CARTESIAN_POINT('Ctrl Pts',(17.3633653656324,17.0470874900869,-12.0385400073471));
#48148=CARTESIAN_POINT('Ctrl Pts',(17.2915493867661,17.096068268624,-12.042856170086));
#48149=CARTESIAN_POINT('Ctrl Pts',(17.2220728058576,17.1434535034522,-12.0470317342777));
#48150=CARTESIAN_POINT('Ctrl Pts',(17.1549836708367,17.1942316733332,-12.0512072984694));
#48151=CARTESIAN_POINT('Ctrl Pts',(17.0906175572635,17.2481209545911,-12.055382862661));
#48152=CARTESIAN_POINT('Ctrl Pts',(17.0230004643096,17.3047320553358,-12.0597693246736));
#48153=CARTESIAN_POINT('Ctrl Pts',(16.9583891293618,17.3647764140015,-12.0641557866861));
#48154=CARTESIAN_POINT('Ctrl Pts',(16.897128197962,17.427884192522,-12.0685422486987));
#48155=CARTESIAN_POINT('Ctrl Pts',(16.8358672665622,17.4909919710426,-12.0729287107112));
#48156=CARTESIAN_POINT('Ctrl Pts',(16.7779570635865,17.5571626827012,-12.0773151727237));
#48157=CARTESIAN_POINT('Ctrl Pts',(16.7236914224212,17.6259891410741,-12.0817016347363));
#48158=CARTESIAN_POINT('Ctrl Pts',(16.6719732357611,17.6915845997261,-12.0858821780095));
#48159=CARTESIAN_POINT('Ctrl Pts',(16.62336875941,17.759841108002,-12.0900627212828));
#48160=CARTESIAN_POINT('Ctrl Pts',(16.5781640651477,17.8304307616062,-12.094243264556));
#48161=CARTESIAN_POINT('Ctrl Pts',(16.5330221281563,17.9009224162283,-12.0984180040186));
#48162=CARTESIAN_POINT('Ctrl Pts',(16.4912708487475,17.9737404018919,-12.1025927434812));
#48163=CARTESIAN_POINT('Ctrl Pts',(16.4531558825329,18.0485241457064,-12.1067674829438));
#48164=CARTESIAN_POINT('Ctrl Pts',(16.4150823671077,18.1232265607011,-12.1109376822935));
#48165=CARTESIAN_POINT('Ctrl Pts',(16.3806375190246,18.1998900805266,-12.1151078816433));
#48166=CARTESIAN_POINT('Ctrl Pts',(16.350022764859,18.2781267276155,-12.1192780809931));
#48167=CARTESIAN_POINT('Ctrl Pts',(16.3194306012405,18.3563056440868,-12.1234452031636));
#48168=CARTESIAN_POINT('Ctrl Pts',(16.2926630858421,18.4360549550053,-12.1276123253342));
#48169=CARTESIAN_POINT('Ctrl Pts',(16.2698743296475,18.5169649283287,-12.1317794475047));
#48170=CARTESIAN_POINT('Ctrl Pts',(16.2470959536793,18.597838047344,-12.1359446715606));
#48171=CARTESIAN_POINT('Ctrl Pts',(16.2282928589741,18.6798703351889,-12.1401098956165));
#48172=CARTESIAN_POINT('Ctrl Pts',(16.2135694673997,18.7626363860258,-12.1442751196725));
#48173=CARTESIAN_POINT('Ctrl Pts',(16.1988435352844,18.8454167182549,-12.1484410624433));
#48174=CARTESIAN_POINT('Ctrl Pts',(16.1881988016352,18.9289306143268,-12.1526070052142));
#48175=CARTESIAN_POINT('Ctrl Pts',(16.181688476361,19.0127428783137,-12.1567729479851));
#48176=CARTESIAN_POINT('Ctrl Pts',(16.1765121589546,19.0793814658902,-12.1600852620662));
#48177=CARTESIAN_POINT('Ctrl Pts',(16.1739485082683,19.146208402676,-12.1633975761474));
#48178=CARTESIAN_POINT('Ctrl Pts',(16.1740007840082,19.2130035272629,-12.1667098902285));
#48179=CARTESIAN_POINT('Origin',(18.734,19.211,1.76670989022852));
#48180=CARTESIAN_POINT('',(20.2922820246455,21.2395345685085,-10.8502164908111));
#48181=CARTESIAN_POINT('',(20.294805058443,21.242816933186,-10.916593671796));
#48182=CARTESIAN_POINT('',(20.2935358855687,21.2411349269503,1.76670989022852));
#48183=CARTESIAN_POINT('',(16.1739804710165,19.212301045312,-11.4332901033202));
#48184=CARTESIAN_POINT('Ctrl Pts',(20.2948050584429,21.242816933186,-10.916593671796));
#48185=CARTESIAN_POINT('Ctrl Pts',(20.3968578837659,21.1659198988778,-10.9229640541024));
#48186=CARTESIAN_POINT('Ctrl Pts',(21.1313726010512,20.5183599193142,-10.9717263719693));
#48187=CARTESIAN_POINT('Ctrl Pts',(21.6797114024885,18.5138092582024,-11.0628806253966));
#48188=CARTESIAN_POINT('Ctrl Pts',(19.7422306313066,16.3567467541765,-11.1900564320781));
#48189=CARTESIAN_POINT('Ctrl Pts',(16.9631832240595,16.8048336241861,-11.3135258905591));
#48190=CARTESIAN_POINT('Ctrl Pts',(16.1754043777096,18.4373668536376,-11.3946034134798));
#48191=CARTESIAN_POINT('Ctrl Pts',(16.1705865747788,19.2122806865248,-11.4332890008399));
#48192=CARTESIAN_POINT('Ctrl Pts',(16.1740003306697,19.212301164443,-11.4332901097715));
#48193=CARTESIAN_POINT('Ctrl Pts',(16.174038011382,19.2864367677247,-11.436996088328));
#48194=CARTESIAN_POINT('Ctrl Pts',(16.1772957565522,19.3604881810636,-11.4407020668845));
#48195=CARTESIAN_POINT('Ctrl Pts',(16.1837535357011,19.4342553948533,-11.444408045441));
#48196=CARTESIAN_POINT('Ctrl Pts',(16.1910453870482,19.5175502156942,-11.448592679834));
#48197=CARTESIAN_POINT('Ctrl Pts',(16.2024358975503,19.6006424250678,-11.4527773142271));
#48198=CARTESIAN_POINT('Ctrl Pts',(16.217906819526,19.6830965019697,-11.4569619486201));
#48199=CARTESIAN_POINT('Ctrl Pts',(16.2333557205591,19.765433215699,-11.4611406267041));
#48200=CARTESIAN_POINT('Ctrl Pts',(16.2528734125179,19.8471331528557,-11.465319304788));
#48201=CARTESIAN_POINT('Ctrl Pts',(16.2763898192683,19.927765093712,-11.4694979828719));
#48202=CARTESIAN_POINT('Ctrl Pts',(16.3003277407088,20.0098423041589,-11.4737515607574));
#48203=CARTESIAN_POINT('Ctrl Pts',(16.3284090988417,20.0908123737401,-11.4780051386428));
#48204=CARTESIAN_POINT('Ctrl Pts',(16.3605053261111,20.1702304379142,-11.4822587165282));
#48205=CARTESIAN_POINT('Ctrl Pts',(16.3919793053844,20.2481088279428,-11.4864298305062));
#48206=CARTESIAN_POINT('Ctrl Pts',(16.4273136905277,20.3244944066986,-11.4906009444841));
#48207=CARTESIAN_POINT('Ctrl Pts',(16.4663372697809,20.3989838980285,-11.4947720584621));
#48208=CARTESIAN_POINT('Ctrl Pts',(16.5053477542952,20.4734483936902,-11.4989417727825));
#48209=CARTESIAN_POINT('Ctrl Pts',(16.5480447610381,20.5460176583688,-11.5031114871028));
#48210=CARTESIAN_POINT('Ctrl Pts',(16.5942102750742,20.6163113296,-11.5072812014232));
#48211=CARTESIAN_POINT('Ctrl Pts',(16.6403741463432,20.6866024994807,-11.5114507673673));
#48212=CARTESIAN_POINT('Ctrl Pts',(16.6900060262588,20.7546178528607,-11.5156203333113));
#48213=CARTESIAN_POINT('Ctrl Pts',(16.7428443053794,20.8200055934583,-11.5197898992554));
#48214=CARTESIAN_POINT('Ctrl Pts',(16.7975403132109,20.8876922863507,-11.5241060619943));
#48215=CARTESIAN_POINT('Ctrl Pts',(16.8556720579015,20.9525627446115,-11.5284222247332));
#48216=CARTESIAN_POINT('Ctrl Pts',(16.916904887788,21.0142651921377,-11.5327383874721));
#48217=CARTESIAN_POINT('Ctrl Pts',(16.9761430646815,21.0739576889257,-11.5369139516638));
#48218=CARTESIAN_POINT('Ctrl Pts',(17.0382830139766,21.1306851185866,-11.5410895158555));
#48219=CARTESIAN_POINT('Ctrl Pts',(17.1029865459478,21.1841687998498,-11.5452650800472));
#48220=CARTESIAN_POINT('Ctrl Pts',(17.1709580995008,21.2403538147083,-11.5496515420597));
#48221=CARTESIAN_POINT('Ctrl Pts',(17.2417585461138,21.2929584378007,-11.5540380040722));
#48222=CARTESIAN_POINT('Ctrl Pts',(17.3149615008576,21.3417110873959,-11.5584244660848));
#48223=CARTESIAN_POINT('Ctrl Pts',(17.3881644556013,21.390463736991,-11.5628109280973));
#48224=CARTESIAN_POINT('Ctrl Pts',(17.4637693807619,21.4353641822178,-11.5671973901099));
#48225=CARTESIAN_POINT('Ctrl Pts',(17.5413224142637,21.4761976020829,-11.5715838521224));
#48226=CARTESIAN_POINT('Ctrl Pts',(17.6153071177329,21.5151522157705,-11.5757684865154));
#48227=CARTESIAN_POINT('Ctrl Pts',(17.6913399834856,21.5505508359911,-11.5799531209085));
#48228=CARTESIAN_POINT('Ctrl Pts',(17.7690449301557,21.5821730668978,-11.5841377553015));
#48229=CARTESIAN_POINT('Ctrl Pts',(17.8466392734521,21.6137502874729,-11.5883164333855));
#48230=CARTESIAN_POINT('Ctrl Pts',(17.9259005477805,21.6415616236984,-11.5924951114694));
#48231=CARTESIAN_POINT('Ctrl Pts',(18.0064282347094,21.6654325874532,-11.5966737895534));
#48232=CARTESIAN_POINT('Ctrl Pts',(18.0883993225523,21.6897314210775,-11.6009273674388));
#48233=CARTESIAN_POINT('Ctrl Pts',(18.1716822438311,21.7099470058045,-11.6051809453242));
#48234=CARTESIAN_POINT('Ctrl Pts',(18.2558333466883,21.7259466498637,-11.6094345232097));
#48235=CARTESIAN_POINT('Ctrl Pts',(18.3383530162092,21.7416361096021,-11.6136056371876));
#48236=CARTESIAN_POINT('Ctrl Pts',(18.4217070321714,21.7532715484977,-11.6177767511656));
#48237=CARTESIAN_POINT('Ctrl Pts',(18.5054636294713,21.7607786428131,-11.6219478651435));
#48238=CARTESIAN_POINT('Ctrl Pts',(18.589192121436,21.7682832180504,-11.6261175794639));
#48239=CARTESIAN_POINT('Ctrl Pts',(18.6733224686327,21.7716621589129,-11.6302872937843));
#48240=CARTESIAN_POINT('Ctrl Pts',(18.7574168390729,21.7708928984721,-11.6344570081046));
#48241=CARTESIAN_POINT('Ctrl Pts',(18.8415082170745,21.7701236654049,-11.6386265740487));
#48242=CARTESIAN_POINT('Ctrl Pts',(18.9255631608593,21.7652065295826,-11.6427961399927));
#48243=CARTESIAN_POINT('Ctrl Pts',(19.0091442611983,21.75617104249,-11.6469657059368));
#48244=CARTESIAN_POINT('Ctrl Pts',(19.095663969917,21.7468178788177,-11.6512818686757));
#48245=CARTESIAN_POINT('Ctrl Pts',(19.1816753701872,21.7330514297719,-11.6555980314146));
#48246=CARTESIAN_POINT('Ctrl Pts',(19.2667015333779,21.7149626747092,-11.6599141941535));
#48247=CARTESIAN_POINT('Ctrl Pts',(19.3489579782457,21.6974631589401,-11.6640897583452));
#48248=CARTESIAN_POINT('Ctrl Pts',(19.4302919452563,21.6759187771978,-11.6682653225369));
#48249=CARTESIAN_POINT('Ctrl Pts',(19.510286051879,21.6504630486355,-11.6724408867286));
#48250=CARTESIAN_POINT('Ctrl Pts',(19.5943204706596,21.6237216117387,-11.6768273487411));
#48251=CARTESIAN_POINT('Ctrl Pts',(19.6768755727334,21.5926635253051,-11.6812138107537));
#48252=CARTESIAN_POINT('Ctrl Pts',(19.757492206768,21.557500309543,-11.6856002727662));
#48253=CARTESIAN_POINT('Ctrl Pts',(19.8381088408025,21.5223370937809,-11.6899867347787));
#48254=CARTESIAN_POINT('Ctrl Pts',(19.9167865216175,21.4830690758565,-11.6943731967913));
#48255=CARTESIAN_POINT('Ctrl Pts',(19.9930989518204,21.4399616034209,-11.6987596588038));
#48256=CARTESIAN_POINT('Ctrl Pts',(20.0658940459184,21.3988410087297,-11.7029439432528));
#48257=CARTESIAN_POINT('Ctrl Pts',(20.1368080586073,21.3540740524687,-11.7071282277018));
#48258=CARTESIAN_POINT('Ctrl Pts',(20.2054522028114,21.3058576120685,-11.7113125121507));
#48259=CARTESIAN_POINT('Ctrl Pts',(20.2352510799466,21.2849265363003,-11.7131289377124));
#48260=CARTESIAN_POINT('Ctrl Pts',(20.2646224642289,21.2633460211763,-11.7149453632741));
#48261=CARTESIAN_POINT('Ctrl Pts',(20.2935358855687,21.2411349269503,-11.7167617888358));
#48262=CARTESIAN_POINT('',(16.1740004874608,19.2094201902091,-11.3667098902285));
#48263=CARTESIAN_POINT('Ctrl Pts',(16.1740004874608,19.2094201902091,-11.3667098902285));
#48264=CARTESIAN_POINT('Ctrl Pts',(16.1739481146197,19.2942876523606,-11.3709134538372));
#48265=CARTESIAN_POINT('Ctrl Pts',(16.1781202862138,19.3791700299234,-11.3751170174459));
#48266=CARTESIAN_POINT('Ctrl Pts',(16.1864949217896,19.463622003183,-11.3793205810546));
#48267=CARTESIAN_POINT('Ctrl Pts',(16.1948707822013,19.5480863280015,-11.3835247594573));
#48268=CARTESIAN_POINT('Ctrl Pts',(16.2074502833288,19.6321196761629,-11.3877289378599));
#48269=CARTESIAN_POINT('Ctrl Pts',(16.2241595327125,19.7152824890538,-11.3919331162626));
#48270=CARTESIAN_POINT('Ctrl Pts',(16.2408759290273,19.7984808725962,-11.3961390928892));
#48271=CARTESIAN_POINT('Ctrl Pts',(16.2617254950327,19.8808075406061,-11.4003450695159));
#48272=CARTESIAN_POINT('Ctrl Pts',(16.2865836343726,19.9618349574034,-11.4045510461425));
#48273=CARTESIAN_POINT('Ctrl Pts',(16.3114761780105,20.0429745182097,-11.408762843948));
#48274=CARTESIAN_POINT('Ctrl Pts',(16.3403882340966,20.1228108093805,-11.4129746417534));
#48275=CARTESIAN_POINT('Ctrl Pts',(16.3731460171587,20.200933569338,-11.4171864395589));
#48276=CARTESIAN_POINT('Ctrl Pts',(16.4059305542806,20.27912013401,-11.4214016772397));
#48277=CARTESIAN_POINT('Ctrl Pts',(16.4425668768386,20.3555899771936,-11.4256169149205));
#48278=CARTESIAN_POINT('Ctrl Pts',(16.4828349986459,20.4299569872143,-11.4298321526013));
#48279=CARTESIAN_POINT('Ctrl Pts',(16.5231739006092,20.5044547137505,-11.4340547994973));
#48280=CARTESIAN_POINT('Ctrl Pts',(16.5671571084148,20.5768418481604,-11.4382774463933));
#48281=CARTESIAN_POINT('Ctrl Pts',(16.6145212917448,20.646761124022,-11.4425000932893));
#48282=CARTESIAN_POINT('Ctrl Pts',(16.6269438222718,20.6650993339888,-11.4436075959693));
#48283=CARTESIAN_POINT('Ctrl Pts',(16.6395987151329,20.6832679625289,-11.4447150986492));
#48284=CARTESIAN_POINT('Ctrl Pts',(16.6524807786036,20.7012609606902,-11.4458226013291));
#48285=CARTESIAN_POINT('Ctrl Pts',(16.7011549053849,20.7692464566217,-11.4500072357222));
#48286=CARTESIAN_POINT('Ctrl Pts',(16.7532538754925,20.8349713096213,-11.4541918701152));
#48287=CARTESIAN_POINT('Ctrl Pts',(16.8085402991528,20.8980699275411,-11.4583765045082));
#48288=CARTESIAN_POINT('Ctrl Pts',(16.8637480294321,20.9610787323883,-11.4625551825922));
#48289=CARTESIAN_POINT('Ctrl Pts',(16.9221339008884,21.0214683841931,-11.4667338606761));
#48290=CARTESIAN_POINT('Ctrl Pts',(16.9834181011141,21.0789033741853,-11.4709125387601));
#48291=CARTESIAN_POINT('Ctrl Pts',(17.0458007765846,21.1373678450953,-11.4751661166455));
#48292=CARTESIAN_POINT('Ctrl Pts',(17.1111864272472,21.1927702956729,-11.479419694531));
#48293=CARTESIAN_POINT('Ctrl Pts',(17.1792379481545,21.2447932446887,-11.4836732724164));
#48294=CARTESIAN_POINT('Ctrl Pts',(17.2459701575374,21.2958076273233,-11.4878443863943));
#48295=CARTESIAN_POINT('Ctrl Pts',(17.3152654110889,21.3435720832561,-11.4920155003723));
#48296=CARTESIAN_POINT('Ctrl Pts',(17.3867710660548,21.3878266351598,-11.4961866143502));
#48297=CARTESIAN_POINT('Ctrl Pts',(17.4582527266078,21.4320663370212,-11.5003563286706));
#48298=CARTESIAN_POINT('Ctrl Pts',(17.5319429246536,21.4727982320514,-11.504526042991));
#48299=CARTESIAN_POINT('Ctrl Pts',(17.6074603942082,21.5098058892787,-11.5086957573114));
#48300=CARTESIAN_POINT('Ctrl Pts',(17.6829751765272,21.5468122296147,-11.5128653232554));
#48301=CARTESIAN_POINT('Ctrl Pts',(17.7603166876031,21.5800943939659,-11.5170348891995));
#48302=CARTESIAN_POINT('Ctrl Pts',(17.8390806772785,21.6094827299398,-11.5212044551435));
#48303=CARTESIAN_POINT('Ctrl Pts',(17.9206139116649,21.6399043235521,-11.5255206178824));
#48304=CARTESIAN_POINT('Ctrl Pts',(18.0036710203273,21.6661529958308,-11.5298367806213));
#48305=CARTESIAN_POINT('Ctrl Pts',(18.0877848913439,21.6880962906889,-11.5341529433603));
#48306=CARTESIAN_POINT('Ctrl Pts',(18.1691587618594,21.709324785025,-11.5383285075519));
#48307=CARTESIAN_POINT('Ctrl Pts',(18.2515211332009,21.7265240396989,-11.5425040717436));
#48308=CARTESIAN_POINT('Ctrl Pts',(18.3344390537293,21.7396263168399,-11.5466796359353));
#48309=CARTESIAN_POINT('Ctrl Pts',(18.4215449613048,21.7533903588515,-11.5510660979478));
#48310=CARTESIAN_POINT('Ctrl Pts',(18.5092634338797,21.7626326086007,-11.5554525599604));
#48311=CARTESIAN_POINT('Ctrl Pts',(18.5970892183629,21.7673363311332,-11.5598390219729));
#48312=CARTESIAN_POINT('Ctrl Pts',(18.6849150028461,21.7720400536657,-11.5642254839854));
#48313=CARTESIAN_POINT('Ctrl Pts',(18.7728475188788,21.7722053239559,-11.568611945998));
#48314=CARTESIAN_POINT('Ctrl Pts',(18.8603867536229,21.7678782506229,-11.5729984080105));
#48315=CARTESIAN_POINT('Ctrl Pts',(18.9438873685616,21.7637508066803,-11.5771825007379));
#48316=CARTESIAN_POINT('Ctrl Pts',(19.0273409554121,21.7555210317051,-11.5813665934653));
#48317=CARTESIAN_POINT('Ctrl Pts',(19.1103117838489,21.7431906407963,-11.5855506861926));
#48318=CARTESIAN_POINT('Ctrl Pts',(19.1931709965624,21.7308768372295,-11.5897291503088));
#48319=CARTESIAN_POINT('Ctrl Pts',(19.2755482894351,21.7144734377188,-11.5939076144249));
#48320=CARTESIAN_POINT('Ctrl Pts',(19.3570101615098,21.6940340993743,-11.5980860785411));
#48321=CARTESIAN_POINT('Ctrl Pts',(19.4414693000141,21.6728427264754,-11.6024182829274));
#48322=CARTESIAN_POINT('Ctrl Pts',(19.5249438445757,21.6473126685892,-11.6067504873137));
#48323=CARTESIAN_POINT('Ctrl Pts',(19.6069591087771,21.6175623603811,-11.6110826917));
#48324=CARTESIAN_POINT('Ctrl Pts',(19.6859209478749,21.5889196549931,-11.6152536082852));
#48325=CARTESIAN_POINT('Ctrl Pts',(19.7635297647264,21.5563655402172,-11.6194245248703));
#48326=CARTESIAN_POINT('Ctrl Pts',(19.8393764665943,21.520056705042,-11.6235954414554));
#48327=CARTESIAN_POINT('Ctrl Pts',(19.9151926435138,21.4837624825697,-11.6277646794308));
#48328=CARTESIAN_POINT('Ctrl Pts',(19.9892477014193,21.4437167433873,-11.6319339174062));
#48329=CARTESIAN_POINT('Ctrl Pts',(20.0611538610254,21.4001237126223,-11.6361031553816));
#48330=CARTESIAN_POINT('Ctrl Pts',(20.1330612495339,21.3565299368366,-11.6402724646108));
#48331=CARTESIAN_POINT('Ctrl Pts',(20.2028192725658,21.3093889858049,-11.64444177384));
#48332=CARTESIAN_POINT('Ctrl Pts',(20.2700670841355,21.2589496851816,-11.6486110830691));
#48333=CARTESIAN_POINT('Ctrl Pts',(20.2779244358431,21.2530562692379,-11.6490982324384));
#48334=CARTESIAN_POINT('Ctrl Pts',(20.2857475522636,21.2471178717865,-11.6495853818077));
#48335=CARTESIAN_POINT('Ctrl Pts',(20.2935358855687,21.2411349269503,-11.650072531177));
#48336=CARTESIAN_POINT('Ctrl Pts',(20.2922820246457,21.2395345685083,-10.8502164908111));
#48337=CARTESIAN_POINT('Ctrl Pts',(20.7519191422662,20.8801556606603,-10.8791841187419));
#48338=CARTESIAN_POINT('Ctrl Pts',(21.5989576388621,19.6129801404785,-10.9505436822331));
#48339=CARTESIAN_POINT('Ctrl Pts',(20.9146849580311,17.1114988461662,-11.0642951812848));
#48340=CARTESIAN_POINT('Ctrl Pts',(18.1490151907075,16.2409688967909,-11.1914709879662));
#48341=CARTESIAN_POINT('Ctrl Pts',(16.3822353164858,17.7107520392007,-11.2922755723079));
#48342=CARTESIAN_POINT('Ctrl Pts',(16.1753926962513,18.8863578053553,-11.3506882210889));
#48343=CARTESIAN_POINT('Ctrl Pts',(16.1772046638934,19.209402892261,-11.3667089343096));
#48344=CARTESIAN_POINT('Origin',(18.734,19.211,1.76670989022852));
#48345=CARTESIAN_POINT('',(20.2935358855687,21.2411349269503,-10.0501312779792));
#48346=CARTESIAN_POINT('',(20.2935358855687,21.2411349269503,-10.1166694969415));
#48347=CARTESIAN_POINT('',(20.2935358855687,21.2411349269503,1.76670989022852));
#48348=CARTESIAN_POINT('',(16.1740004874608,19.2125798097913,-10.6332901097715));
#48349=CARTESIAN_POINT('Ctrl Pts',(20.2935358855687,21.2411349269503,-10.1166694969415));
#48350=CARTESIAN_POINT('Ctrl Pts',(20.3602256392546,21.1899043103582,-10.1208396570584));
#48351=CARTESIAN_POINT('Ctrl Pts',(20.4243735057776,21.1353955467902,-10.1250098171752));
#48352=CARTESIAN_POINT('Ctrl Pts',(20.485652031861,21.0778998792858,-10.1291799772921));
#48353=CARTESIAN_POINT('Ctrl Pts',(20.5469978512285,21.0203410726601,-10.1333547168887));
#48354=CARTESIAN_POINT('Ctrl Pts',(20.6054677052745,20.9597891308285,-10.1375294564853));
#48355=CARTESIAN_POINT('Ctrl Pts',(20.6607708292776,20.8965723572261,-10.1417041960819));
#48356=CARTESIAN_POINT('Ctrl Pts',(20.7161082312277,20.8333164006436,-10.1458815232629));
#48357=CARTESIAN_POINT('Ctrl Pts',(20.7682747110444,20.7673926852028,-10.150058850444));
#48358=CARTESIAN_POINT('Ctrl Pts',(20.817021149451,20.6991609089544,-10.154236177625));
#48359=CARTESIAN_POINT('Ctrl Pts',(20.8658480288831,20.6308165371147,-10.1584203982016));
#48360=CARTESIAN_POINT('Ctrl Pts',(20.9112433534327,20.5601568885703,-10.1626046187782));
#48361=CARTESIAN_POINT('Ctrl Pts',(20.953002718353,20.4875684219587,-10.1667888393548));
#48362=CARTESIAN_POINT('Ctrl Pts',(20.9725011688784,20.4536751233502,-10.1687425524454));
#48363=CARTESIAN_POINT('Ctrl Pts',(20.9912075871119,20.4193616240964,-10.170696265536));
#48364=CARTESIAN_POINT('Ctrl Pts',(21.0091047687182,20.3846687315233,-10.1726499786266));
#48365=CARTESIAN_POINT('Ctrl Pts',(21.0474385251168,20.310360445341,-10.1768346130196));
#48366=CARTESIAN_POINT('Ctrl Pts',(21.0821992629534,20.2340338438632,-10.1810192474127));
#48367=CARTESIAN_POINT('Ctrl Pts',(21.1131697431269,20.1560668406994,-10.1852038818057));
#48368=CARTESIAN_POINT('Ctrl Pts',(21.1440961406553,20.0782108139141,-10.1893825598897));
#48369=CARTESIAN_POINT('Ctrl Pts',(21.1712428282377,19.9987194471871,-10.1935612379736));
#48370=CARTESIAN_POINT('Ctrl Pts',(21.194438677507,19.9179947059402,-10.1977399160576));
#48371=CARTESIAN_POINT('Ctrl Pts',(21.218050295704,19.8358230317223,-10.201993493943));
#48372=CARTESIAN_POINT('Ctrl Pts',(21.2375678238504,19.75237376008,-10.2062470718284));
#48373=CARTESIAN_POINT('Ctrl Pts',(21.252862289631,19.668091638378,-10.2105006497139));
#48374=CARTESIAN_POINT('Ctrl Pts',(21.2678602423477,19.5854434900683,-10.2146717636918));
#48375=CARTESIAN_POINT('Ctrl Pts',(21.2787973301571,19.5019949698563,-10.2188428776698));
#48376=CARTESIAN_POINT('Ctrl Pts',(21.2856028472,19.4181784500402,-10.2230139916477));
#48377=CARTESIAN_POINT('Ctrl Pts',(21.2924060805859,19.3343900556667,-10.2271837059681));
#48378=CARTESIAN_POINT('Ctrl Pts',(21.2950804593957,19.2502343650762,-10.2313534202885));
#48379=CARTESIAN_POINT('Ctrl Pts',(21.2936070835643,19.1661493838665,-10.2355231346088));
#48380=CARTESIAN_POINT('Ctrl Pts',(21.2921337601619,19.0820673947614,-10.2396927005529));
#48381=CARTESIAN_POINT('Ctrl Pts',(21.2865129844866,18.9980565699817,-10.2438622664969));
#48382=CARTESIAN_POINT('Ctrl Pts',(21.2767779695197,18.9145540559809,-10.248031832441));
#48383=CARTESIAN_POINT('Ctrl Pts',(21.2667006834359,18.8281156965991,-10.2523479951799));
#48384=CARTESIAN_POINT('Ctrl Pts',(21.2522145228803,18.7422225813446,-10.2566641579188));
#48385=CARTESIAN_POINT('Ctrl Pts',(21.2334144574581,18.6573508603372,-10.2609803206577));
#48386=CARTESIAN_POINT('Ctrl Pts',(21.2152268021896,18.5752438267147,-10.2651558848494));
#48387=CARTESIAN_POINT('Ctrl Pts',(21.1930021468741,18.4940931072451,-10.2693314490411));
#48388=CARTESIAN_POINT('Ctrl Pts',(21.1668775008283,18.4143149518391,-10.2735070132328));
#48389=CARTESIAN_POINT('Ctrl Pts',(21.1394333610162,18.3305073914579,-10.2778934752453));
#48390=CARTESIAN_POINT('Ctrl Pts',(21.1076851096665,18.2482152402674,-10.2822799372578));
#48391=CARTESIAN_POINT('Ctrl Pts',(21.071848104157,18.1678958623945,-10.2866663992704));
#48392=CARTESIAN_POINT('Ctrl Pts',(21.0360110986474,18.0875764845216,-10.2910528612829));
#48393=CARTESIAN_POINT('Ctrl Pts',(20.9960856701952,18.0092303623902,-10.2954393232955));
#48394=CARTESIAN_POINT('Ctrl Pts',(20.9523407266399,17.9332815566288,-10.299825785308));
#48395=CARTESIAN_POINT('Ctrl Pts',(20.9106085527831,17.8608272680037,-10.3040104197011));
#48396=CARTESIAN_POINT('Ctrl Pts',(20.8652452879883,17.7902848467577,-10.3081950540941));
#48397=CARTESIAN_POINT('Ctrl Pts',(20.8164511103896,17.7220415140652,-10.3123796884872));
#48398=CARTESIAN_POINT('Ctrl Pts',(20.7677263852631,17.6538953173098,-10.3165583665711));
#48399=CARTESIAN_POINT('Ctrl Pts',(20.7155807127379,17.5880420799731,-10.3207370446551));
#48400=CARTESIAN_POINT('Ctrl Pts',(20.6602594535819,17.5248432701892,-10.324915722739));
#48401=CARTESIAN_POINT('Ctrl Pts',(20.6039466006143,17.4605116671601,-10.3291693006244));
#48402=CARTESIAN_POINT('Ctrl Pts',(20.5443434371031,17.3989310067054,-10.3334228785099));
#48403=CARTESIAN_POINT('Ctrl Pts',(20.4817541149312,17.3404504674452,-10.3376764563953));
#48404=CARTESIAN_POINT('Ctrl Pts',(20.4203782089026,17.2831036875539,-10.3418475703733));
#48405=CARTESIAN_POINT('Ctrl Pts',(20.3561312476119,17.2287382262735,-10.3460186843512));
#48406=CARTESIAN_POINT('Ctrl Pts',(20.2893385159968,17.1776475709664,-10.3501897983292));
#48407=CARTESIAN_POINT('Ctrl Pts',(20.2225681973279,17.1265740596221,-10.3543595126496));
#48408=CARTESIAN_POINT('Ctrl Pts',(20.1532541699942,17.078773451095,-10.3585292269699));
#48409=CARTESIAN_POINT('Ctrl Pts',(20.0817544971409,17.0344987214715,-10.3626989412903));
#48410=CARTESIAN_POINT('Ctrl Pts',(20.0102573685527,16.9902255673327,-10.3668685072343));
#48411=CARTESIAN_POINT('Ctrl Pts',(19.9365751406475,16.9494782841066,-10.3710380731784));
#48412=CARTESIAN_POINT('Ctrl Pts',(19.8610933619694,16.912465564016,-10.3752076391224));
#48413=CARTESIAN_POINT('Ctrl Pts',(19.78295773707,16.8741515223472,-10.3795238018614));
#48414=CARTESIAN_POINT('Ctrl Pts',(19.7028941360643,16.8398397766944,-10.3838399646003));
#48415=CARTESIAN_POINT('Ctrl Pts',(19.6213543310965,16.8097082036778,-10.3881561273392));
#48416=CARTESIAN_POINT('Ctrl Pts',(19.5424706766991,16.780558163483,-10.3923316915309));
#48417=CARTESIAN_POINT('Ctrl Pts',(19.4622059796066,16.7553202361716,-10.3965072557226));
#48418=CARTESIAN_POINT('Ctrl Pts',(19.3809844006654,16.7341045267723,-10.4006828199142));
#48419=CARTESIAN_POINT('Ctrl Pts',(19.2956605128579,16.7118172623269,-10.4050692819268));
#48420=CARTESIAN_POINT('Ctrl Pts',(19.2092811104196,16.693969336797,-10.4094557439393));
#48421=CARTESIAN_POINT('Ctrl Pts',(19.122347333066,16.6806272312364,-10.4138422059519));
#48422=CARTESIAN_POINT('Ctrl Pts',(19.0354135557124,16.6672851256757,-10.4182286679644));
#48423=CARTESIAN_POINT('Ctrl Pts',(18.9479259883671,16.65844882271,-10.4226151299769));
#48424=CARTESIAN_POINT('Ctrl Pts',(18.8603867536229,16.6541217493771,-10.4270015919895));
#48425=CARTESIAN_POINT('Ctrl Pts',(18.7768753288335,16.6499937711024,-10.4311862263825));
#48426=CARTESIAN_POINT('Ctrl Pts',(18.6930060412947,16.6499538232249,-10.4353708607756));
#48427=CARTESIAN_POINT('Ctrl Pts',(18.6092128353623,16.6540431830902,-10.4395554951686));
#48428=CARTESIAN_POINT('Ctrl Pts',(18.5255388986872,16.6581267222578,-10.4437341732526));
#48429=CARTESIAN_POINT('Ctrl Pts',(18.441941284071,16.6663278722549,-10.4479128513365));
#48430=CARTESIAN_POINT('Ctrl Pts',(18.3588567381408,16.6786359793502,-10.4520915294204));
#48431=CARTESIAN_POINT('Ctrl Pts',(18.2742829614366,16.6911647004195,-10.4563451073059));
#48432=CARTESIAN_POINT('Ctrl Pts',(18.1902413093998,16.7079490849927,-10.4605986851913));
#48433=CARTESIAN_POINT('Ctrl Pts',(18.1071900176367,16.7289223932339,-10.4648522630768));
#48434=CARTESIAN_POINT('Ctrl Pts',(18.0257488372257,16.7494890929688,-10.4690233770547));
#48435=CARTESIAN_POINT('Ctrl Pts',(17.945260426203,16.7740836270436,-10.4731944910327));
#48436=CARTESIAN_POINT('Ctrl Pts',(17.8661476315623,16.8025913414461,-10.4773656050106));
#48437=CARTESIAN_POINT('Ctrl Pts',(17.7870613839839,16.8310894898098,-10.481535319331));
#48438=CARTESIAN_POINT('Ctrl Pts',(17.7093502684716,16.8634980548293,-10.4857050336514));
#48439=CARTESIAN_POINT('Ctrl Pts',(17.633420810669,16.8996528932219,-10.4898747479717));
#48440=CARTESIAN_POINT('Ctrl Pts',(17.5574940547624,16.9358064450701,-10.4940443139158));
#48441=CARTESIAN_POINT('Ctrl Pts',(17.4833492454956,16.975705806696,-10.4982138798598));
#48442=CARTESIAN_POINT('Ctrl Pts',(17.4113705501161,17.0191397539305,-10.5023834458039));
#48443=CARTESIAN_POINT('Ctrl Pts',(17.3368611726025,17.0641007851681,-10.5066996085428));
#48444=CARTESIAN_POINT('Ctrl Pts',(17.2646735157618,17.1128493061263,-10.5110157712817));
#48445=CARTESIAN_POINT('Ctrl Pts',(17.1952016813754,17.1651017291669,-10.5153319340206));
#48446=CARTESIAN_POINT('Ctrl Pts',(17.1279928846869,17.2156520350229,-10.5195074982123));
#48447=CARTESIAN_POINT('Ctrl Pts',(17.0633260236108,17.2694811317355,-10.523683062404));
#48448=CARTESIAN_POINT('Ctrl Pts',(17.001523269273,17.3262919649215,-10.5278586265957));
#48449=CARTESIAN_POINT('Ctrl Pts',(16.9365990047358,17.3859721782367,-10.5322450886082));
#48450=CARTESIAN_POINT('Ctrl Pts',(16.8748361916357,17.4489428422738,-10.5366315506207));
#48451=CARTESIAN_POINT('Ctrl Pts',(16.8165619874411,17.5148185627727,-10.5410180126333));
#48452=CARTESIAN_POINT('Ctrl Pts',(16.7582877832466,17.5806942832717,-10.5454044746458));
#48453=CARTESIAN_POINT('Ctrl Pts',(16.7035024899566,17.6494745589998,-10.5497909366584));
#48454=CARTESIAN_POINT('Ctrl Pts',(16.6524807786037,17.7207390393097,-10.5541773986709));
#48455=CARTESIAN_POINT('Ctrl Pts',(16.6033728384837,17.789330463214,-10.5583993290636));
#48456=CARTESIAN_POINT('Ctrl Pts',(16.5575691753499,17.8604769154311,-10.5626212594564));
#48457=CARTESIAN_POINT('Ctrl Pts',(16.5153433201941,17.9338302629828,-10.5668431898491));
#48458=CARTESIAN_POINT('Ctrl Pts',(16.4731798646834,18.0070752119517,-10.5710588812454));
#48459=CARTESIAN_POINT('Ctrl Pts',(16.4345839361663,18.082520192057,-10.5752745726418));
#48460=CARTESIAN_POINT('Ctrl Pts',(16.3997870211447,18.1597865253224,-10.5794902640381));
#48461=CARTESIAN_POINT('Ctrl Pts',(16.3650317212893,18.2369604523703,-10.5837009137031));
#48462=CARTESIAN_POINT('Ctrl Pts',(16.3340665899183,18.3159509969196,-10.587911563368));
#48463=CARTESIAN_POINT('Ctrl Pts',(16.3070776023613,18.3963542635971,-10.592122213033));
#48464=CARTESIAN_POINT('Ctrl Pts',(16.2801155537106,18.4766772762055,-10.5963286598617));
#48465=CARTESIAN_POINT('Ctrl Pts',(16.2571218975382,18.5584097818784,-10.6005351066903));
#48466=CARTESIAN_POINT('Ctrl Pts',(16.238234292144,18.6411284956326,-10.604741553519));
#48467=CARTESIAN_POINT('Ctrl Pts',(16.2193575415099,18.7237996707085,-10.6089455828908));
#48468=CARTESIAN_POINT('Ctrl Pts',(16.2045822501751,18.807455489948,-10.6131496122625));
#48469=CARTESIAN_POINT('Ctrl Pts',(16.19399578679,18.8916591211959,-10.6173536416343));
#48470=CARTESIAN_POINT('Ctrl Pts',(16.1834116610726,18.975844158877,-10.6215567426863));
#48471=CARTESIAN_POINT('Ctrl Pts',(16.1770145819501,19.0605763228053,-10.6257598437382));
#48472=CARTESIAN_POINT('Ctrl Pts',(16.1748403468596,19.145411359684,-10.6299629447902));
#48473=CARTESIAN_POINT('Ctrl Pts',(16.1742666403856,19.1677964320708,-10.631071999784));
#48474=CARTESIAN_POINT('Ctrl Pts',(16.1739866695752,19.1901886456578,-10.6321810547777));
#48475=CARTESIAN_POINT('Ctrl Pts',(16.1740004874608,19.2125798097913,-10.6332901097715));
#48476=CARTESIAN_POINT('Ctrl Pts',(16.1772048569635,19.2125971087803,-10.6332910657481));
#48477=CARTESIAN_POINT('Ctrl Pts',(16.1753928896008,19.5356421709025,-10.6493117789495));
#48478=CARTESIAN_POINT('Ctrl Pts',(16.3822354944161,20.7112478477878,-10.7077244277114));
#48479=CARTESIAN_POINT('Ctrl Pts',(18.0373629477008,22.0881474066249,-10.8021586297274));
#48480=CARTESIAN_POINT('Ctrl Pts',(19.7177437291103,21.6776339477978,-10.8805721185419));
#48481=CARTESIAN_POINT('Ctrl Pts',(20.2948050584429,21.242816933186,-10.916593671796));
#48482=CARTESIAN_POINT('',(16.1739802642219,19.2096989559289,-10.5667098967469));
#48483=CARTESIAN_POINT('Ctrl Pts',(16.1705863812103,19.2097193146384,-10.566710999223));
#48484=CARTESIAN_POINT('Ctrl Pts',(16.1754041849044,19.9846332056276,-10.6053965865622));
#48485=CARTESIAN_POINT('Ctrl Pts',(16.9631830908079,21.6171665575917,-10.6864741094618));
#48486=CARTESIAN_POINT('Ctrl Pts',(19.0902280311167,21.9601261297055,-10.7809759399911));
#48487=CARTESIAN_POINT('Ctrl Pts',(20.0792749368812,21.4060795485156,-10.8367921831814));
#48488=CARTESIAN_POINT('Ctrl Pts',(20.2922820246457,21.2395345685083,-10.8502164908111));
#48489=CARTESIAN_POINT('Ctrl Pts',(20.2935358855687,21.2411349269503,-10.0501312779792));
#48490=CARTESIAN_POINT('Ctrl Pts',(20.3598784985668,21.1901709814807,-10.0543142410822));
#48491=CARTESIAN_POINT('Ctrl Pts',(20.4238373144014,21.1358617299933,-10.0584972041852));
#48492=CARTESIAN_POINT('Ctrl Pts',(20.4850560901097,21.0784588534395,-10.0626801672881));
#48493=CARTESIAN_POINT('Ctrl Pts',(20.5461929654509,21.0211327722253,-10.066857534294));
#48494=CARTESIAN_POINT('Ctrl Pts',(20.6045967494064,20.9607215996642,-10.0710349012998));
#48495=CARTESIAN_POINT('Ctrl Pts',(20.6599429808172,20.8975181987281,-10.0752122683057));
#48496=CARTESIAN_POINT('Ctrl Pts',(20.7152315969333,20.8343805923813,-10.0793852866824));
#48497=CARTESIAN_POINT('Ctrl Pts',(20.7674686848818,20.7684568792845,-10.0835583050592));
#48498=CARTESIAN_POINT('Ctrl Pts',(20.8163664780353,20.7000768452819,-10.087731323436));
#48499=CARTESIAN_POINT('Ctrl Pts',(20.8652367012063,20.6317353659098,-10.091901988945));
#48500=CARTESIAN_POINT('Ctrl Pts',(20.9107711007099,20.5609406886882,-10.0960726544539));
#48501=CARTESIAN_POINT('Ctrl Pts',(20.9527227999439,20.4880548684411,-10.1002433199629));
#48502=CARTESIAN_POINT('Ctrl Pts',(20.9946634302466,20.4151882790751,-10.1044128850442));
#48503=CARTESIAN_POINT('Ctrl Pts',(21.0330230085846,20.3402320411324,-10.1085824501255));
#48504=CARTESIAN_POINT('Ctrl Pts',(21.0675992698966,20.2635751505417,-10.1127520152067));
#48505=CARTESIAN_POINT('Ctrl Pts',(21.1021767802658,20.1869154907437,-10.1169217309123));
#48506=CARTESIAN_POINT('Ctrl Pts',(21.1329705142616,20.1085554762028,-10.1210914466179));
#48507=CARTESIAN_POINT('Ctrl Pts',(21.1598258280554,20.0289052829879,-10.1252611623235));
#48508=CARTESIAN_POINT('Ctrl Pts',(21.186708599274,19.9491736537782,-10.1294351412322));
#48509=CARTESIAN_POINT('Ctrl Pts',(21.2096447603305,19.8681496481244,-10.1336091201408));
#48510=CARTESIAN_POINT('Ctrl Pts',(21.2285293380277,19.7862594038511,-10.1377830990495));
#48511=CARTESIAN_POINT('Ctrl Pts',(21.2474234553482,19.7043277923787,-10.141959186461));
#48512=CARTESIAN_POINT('Ctrl Pts',(21.2622618315702,19.6215295239771,-10.1461352738725));
#48513=CARTESIAN_POINT('Ctrl Pts',(21.2729909701164,19.5382993334354,-10.150311361284));
#48514=CARTESIAN_POINT('Ctrl Pts',(21.2837392233131,19.4549208629554,-10.1544948886639));
#48515=CARTESIAN_POINT('Ctrl Pts',(21.2903635757193,19.3711093924122,-10.1586784160438));
#48516=CARTESIAN_POINT('Ctrl Pts',(21.2928626077066,19.2873030463401,-10.1628619434237));
#48517=CARTESIAN_POINT('Ctrl Pts',(21.2950932320049,19.2124978926481,-10.166596140454));
#48518=CARTESIAN_POINT('Ctrl Pts',(21.2940378520455,19.1376970537945,-10.1703303374844));
#48519=CARTESIAN_POINT('Ctrl Pts',(21.2897303495757,19.0632083214199,-10.1740645345147));
#48520=CARTESIAN_POINT('Ctrl Pts',(21.2849032547982,18.9797343887762,-10.1782491689078));
#48521=CARTESIAN_POINT('Ctrl Pts',(21.2759733033623,18.8963418534062,-10.1824338033008));
#48522=CARTESIAN_POINT('Ctrl Pts',(21.262945864237,18.8134665853561,-10.1866184376939));
#48523=CARTESIAN_POINT('Ctrl Pts',(21.2499369680589,18.7307092799923,-10.1907971157778));
#48524=CARTESIAN_POINT('Ctrl Pts',(21.2328422397339,18.6484682300579,-10.1949757938618));
#48525=CARTESIAN_POINT('Ctrl Pts',(21.2117189811603,18.5671765378629,-10.1991544719457));
#48526=CARTESIAN_POINT('Ctrl Pts',(21.1902171033576,18.4844277505086,-10.2034080498311));
#48527=CARTESIAN_POINT('Ctrl Pts',(21.1645408797953,18.4026631714651,-10.2076616277166));
#48528=CARTESIAN_POINT('Ctrl Pts',(21.1348056750071,18.3223312704649,-10.211915205602));
#48529=CARTESIAN_POINT('Ctrl Pts',(21.1056469451872,18.2435567601204,-10.21608631958));
#48530=CARTESIAN_POINT('Ctrl Pts',(21.0725853792787,18.1661603243174,-10.2202574335579));
#48531=CARTESIAN_POINT('Ctrl Pts',(21.0357801964354,18.0905501228087,-10.2244285475359));
#48532=CARTESIAN_POINT('Ctrl Pts',(20.9989873639266,18.0149652930333,-10.2285982618562));
#48533=CARTESIAN_POINT('Ctrl Pts',(20.9584536105076,17.9411659204442,-10.2327679761766));
#48534=CARTESIAN_POINT('Ctrl Pts',(20.9143856152223,17.8695386442646,-10.236937690497));
#48535=CARTESIAN_POINT('Ctrl Pts',(20.8703191880655,17.7979139168908,-10.241107256441));
#48536=CARTESIAN_POINT('Ctrl Pts',(20.8227190108795,17.7284615236186,-10.2452768223851));
#48537=CARTESIAN_POINT('Ctrl Pts',(20.7718361823765,17.6615408382932,-10.2494463883291));
#48538=CARTESIAN_POINT('Ctrl Pts',(20.719164376394,17.5922673042273,-10.2537625510681));
#48539=CARTESIAN_POINT('Ctrl Pts',(20.6629751073579,17.5257072400677,-10.258078713807));
#48540=CARTESIAN_POINT('Ctrl Pts',(20.6035924848956,17.462222158071,-10.2623948765459));
#48541=CARTESIAN_POINT('Ctrl Pts',(20.546144245114,17.4008050959428,-10.2665704407376));
#48542=CARTESIAN_POINT('Ctrl Pts',(20.4857078751411,17.3422660512048,-10.2707460049293));
#48543=CARTESIAN_POINT('Ctrl Pts',(20.4226131812576,17.2868935777657,-10.2749215691209));
#48544=CARTESIAN_POINT('Ctrl Pts',(20.3563317243794,17.2287243723288,-10.2793080311335));
#48545=CARTESIAN_POINT('Ctrl Pts',(20.2871168004273,17.1740503939331,-10.283694493146));
#48546=CARTESIAN_POINT('Ctrl Pts',(20.2153865821741,17.1231557064392,-10.2880809551586));
#48547=CARTESIAN_POINT('Ctrl Pts',(20.1436563639208,17.0722610189452,-10.2924674171711));
#48548=CARTESIAN_POINT('Ctrl Pts',(20.0694113820225,17.0251458690141,-10.2968538791836));
#48549=CARTESIAN_POINT('Ctrl Pts',(19.9930989518198,16.9820383965787,-10.3012403411962));
#48550=CARTESIAN_POINT('Ctrl Pts',(19.9202977696528,16.9409143628506,-10.3054249755892));
#48551=CARTESIAN_POINT('Ctrl Pts',(19.8453442312191,16.9032842410815,-10.3096096099823));
#48552=CARTESIAN_POINT('Ctrl Pts',(19.7686077403709,16.8693794450073,-10.3137942443753));
#48553=CARTESIAN_POINT('Ctrl Pts',(19.6919804744194,16.8355229082136,-10.3179729224593));
#48554=CARTESIAN_POINT('Ctrl Pts',(19.6135757141379,16.8053813489309,-10.3221516005432));
#48555=CARTESIAN_POINT('Ctrl Pts',(19.5337886464594,16.7791410153969,-10.3263302786272));
#48556=CARTESIAN_POINT('Ctrl Pts',(19.4525714529348,16.752430342743,-10.3305838565126));
#48557=CARTESIAN_POINT('Ctrl Pts',(19.3699223286582,16.7297623675601,-10.334837434398));
#48558=CARTESIAN_POINT('Ctrl Pts',(19.2862808103369,16.7112828346924,-10.3390910122835));
#48559=CARTESIAN_POINT('Ctrl Pts',(19.2042608460612,16.6931615636291,-10.3432621262614));
#48560=CARTESIAN_POINT('Ctrl Pts',(19.1212870932384,16.6790678856914,-10.3474332402394));
#48561=CARTESIAN_POINT('Ctrl Pts',(19.0377889319358,16.6690888519003,-10.3516043542173));
#48562=CARTESIAN_POINT('Ctrl Pts',(18.9543187892476,16.6591131666705,-10.3557740685377));
#48563=CARTESIAN_POINT('Ctrl Pts',(18.8703250439618,16.6532494380237,-10.3599437828581));
#48564=CARTESIAN_POINT('Ctrl Pts',(18.7862446699247,16.6515331620698,-10.3641134971784));
#48565=CARTESIAN_POINT('Ctrl Pts',(18.7021672878281,16.6498169471884,-10.3682830631225));
#48566=CARTESIAN_POINT('Ctrl Pts',(18.6180037430638,16.652247900101,-10.3724526290665));
#48567=CARTESIAN_POINT('Ctrl Pts',(18.5341921271337,16.6588094087744,-10.3766221950106));
#48568=CARTESIAN_POINT('Ctrl Pts',(18.4474337981803,16.6656016119982,-10.3809383577495));
#48569=CARTESIAN_POINT('Ctrl Pts',(18.361053131965,16.6768201947949,-10.3852545204884));
#48570=CARTESIAN_POINT('Ctrl Pts',(18.2755295374795,16.6923883119869,-10.3895706832273));
#48571=CARTESIAN_POINT('Ctrl Pts',(18.1927918650888,16.7074492993989,-10.393746247419));
#48572=CARTESIAN_POINT('Ctrl Pts',(18.1108567316689,16.7265806476473,-10.3979218116107));
#48573=CARTESIAN_POINT('Ctrl Pts',(18.030145283277,16.749661230601,-10.4020973758024));
#48574=CARTESIAN_POINT('Ctrl Pts',(17.9453572914999,16.7739075589308,-10.4064838378149));
#48575=CARTESIAN_POINT('Ctrl Pts',(17.8619204024433,16.8025123689437,-10.4108702998274));
#48576=CARTESIAN_POINT('Ctrl Pts',(17.7802998178505,16.8352778018952,-10.41525676184));
#48577=CARTESIAN_POINT('Ctrl Pts',(17.6986792332576,16.8680432348467,-10.4196432238525));
#48578=CARTESIAN_POINT('Ctrl Pts',(17.6188754477656,16.9049689780518,-10.4240296858651));
#48579=CARTESIAN_POINT('Ctrl Pts',(17.5413224142637,16.9458023979171,-10.4284161478776));
#48580=CARTESIAN_POINT('Ctrl Pts',(17.4673377107945,16.9847570116046,-10.4326007822707));
#48581=CARTESIAN_POINT('Ctrl Pts',(17.3951258047347,17.0274126045708,-10.4367854166637));
#48582=CARTESIAN_POINT('Ctrl Pts',(17.3250812297131,17.0735838265015,-10.4409700510568));
#48583=CARTESIAN_POINT('Ctrl Pts',(17.2551363544742,17.1196893294125,-10.4451487291407));
#48584=CARTESIAN_POINT('Ctrl Pts',(17.1873530634461,17.1693002706272,-10.4493274072246));
#48585=CARTESIAN_POINT('Ctrl Pts',(17.1221018691139,17.2221851731129,-10.4535060853086));
#48586=CARTESIAN_POINT('Ctrl Pts',(17.0556810940185,17.276017999468,-10.457759663194));
#48587=CARTESIAN_POINT('Ctrl Pts',(16.9918845107683,17.3332430884428,-10.4620132410795));
#48588=CARTESIAN_POINT('Ctrl Pts',(16.9310725805955,17.3935697481445,-10.4662668189649));
#48589=CARTESIAN_POINT('Ctrl Pts',(16.8714396083539,17.4527268578301,-10.4704379329429));
#48590=CARTESIAN_POINT('Ctrl Pts',(16.8146769368999,17.5148660125131,-10.4746090469208));
#48591=CARTESIAN_POINT('Ctrl Pts',(16.7610901776527,17.5796732905743,-10.4787801608988));
#48592=CARTESIAN_POINT('Ctrl Pts',(16.7075213999602,17.6444588219275,-10.4829498752191));
#48593=CARTESIAN_POINT('Ctrl Pts',(16.6571267108676,17.7119103443124,-10.4871195895395));
#48594=CARTESIAN_POINT('Ctrl Pts',(16.610172482641,17.7816796452478,-10.4912893038599));
#48595=CARTESIAN_POINT('Ctrl Pts',(16.5632199252474,17.8514464634922,-10.4954588698039));
#48596=CARTESIAN_POINT('Ctrl Pts',(16.5197078414472,17.9235305141742,-10.499628435748));
#48597=CARTESIAN_POINT('Ctrl Pts',(16.4798593937703,17.9975544398918,-10.503798001692));
#48598=CARTESIAN_POINT('Ctrl Pts',(16.4386099238315,18.0741809555191,-10.5081141644309));
#48599=CARTESIAN_POINT('Ctrl Pts',(16.4012867603008,18.1528858318599,-10.5124303271698));
#48600=CARTESIAN_POINT('Ctrl Pts',(16.3680847835396,18.2332243669834,-10.5167464899088));
#48601=CARTESIAN_POINT('Ctrl Pts',(16.3359643576791,18.3109458827753,-10.5209220541004));
#48602=CARTESIAN_POINT('Ctrl Pts',(16.3077008602571,18.3901957994176,-10.5250976182921));
#48603=CARTESIAN_POINT('Ctrl Pts',(16.2834204017388,18.4705544364466,-10.5292731824838));
#48604=CARTESIAN_POINT('Ctrl Pts',(16.2579135949821,18.5549717971974,-10.5336596444963));
#48605=CARTESIAN_POINT('Ctrl Pts',(16.236802907853,18.6406122578469,-10.5380461065089));
#48606=CARTESIAN_POINT('Ctrl Pts',(16.2201737773398,18.726977560163,-10.5424325685214));
#48607=CARTESIAN_POINT('Ctrl Pts',(16.2035446468265,18.8133428624791,-10.546819030534));
#48608=CARTESIAN_POINT('Ctrl Pts',(16.1913970777482,18.9004324212999,-10.5512054925465));
#48609=CARTESIAN_POINT('Ctrl Pts',(16.1837535357011,18.9877446051473,-10.555591954559));
#48610=CARTESIAN_POINT('Ctrl Pts',(16.1772957565522,19.0615118189368,-10.5592979331155));
#48611=CARTESIAN_POINT('Ctrl Pts',(16.174038011382,19.1355632322755,-10.563003911672));
#48612=CARTESIAN_POINT('Ctrl Pts',(16.1740003306697,19.2096988355574,-10.5667098902285));
#48613=CARTESIAN_POINT('Origin',(18.734,19.211,1.76670989022852));
#48614=CARTESIAN_POINT('',(20.2935358855687,21.2411349269503,-9.25004024781016));
#48615=CARTESIAN_POINT('',(20.2929505577762,21.2403915309055,-9.31680761603243));
#48616=CARTESIAN_POINT('',(20.2935358855687,21.2411349269503,1.76670989022852));
#48617=CARTESIAN_POINT('',(16.1740007840082,19.2089964727374,-9.83329010977151));
#48618=CARTESIAN_POINT('Ctrl Pts',(20.2929505577765,21.2403915309053,-9.31680761603245));
#48619=CARTESIAN_POINT('Ctrl Pts',(20.7827497205508,20.8565253562616,-9.34773679020097));
#48620=CARTESIAN_POINT('Ctrl Pts',(21.628276822644,19.5224825845314,-9.42105789992997));
#48621=CARTESIAN_POINT('Ctrl Pts',(20.8151679973455,17.0128120271405,-9.53677094521944));
#48622=CARTESIAN_POINT('Ctrl Pts',(18.012168550104,16.271229608432,-9.66394675190087));
#48623=CARTESIAN_POINT('Ctrl Pts',(16.3483940920526,17.7909994706266,-9.76278617059815));
#48624=CARTESIAN_POINT('Ctrl Pts',(16.1742904286681,18.9257985710608,-9.81923365373494));
#48625=CARTESIAN_POINT('Ctrl Pts',(16.1763511750307,19.2089800092947,-9.83328920131125));
#48626=CARTESIAN_POINT('Ctrl Pts',(16.1740007840082,19.2089964727374,-9.83329010977151));
#48627=CARTESIAN_POINT('Ctrl Pts',(16.1739350379054,19.2930033015151,-9.83745593779553));
#48628=CARTESIAN_POINT('Ctrl Pts',(16.1780086491546,19.3770604200798,-9.84162176581954));
#48629=CARTESIAN_POINT('Ctrl Pts',(16.186209790272,19.4607299485725,-9.84578759384356));
#48630=CARTESIAN_POINT('Ctrl Pts',(16.1944094741073,19.544384609609,-9.84995268163076));
#48631=CARTESIAN_POINT('Ctrl Pts',(16.2067351859308,19.6276513592373,-9.85411776941796));
#48632=CARTESIAN_POINT('Ctrl Pts',(16.2231231591268,19.7100966739689,-9.85828285720516));
#48633=CARTESIAN_POINT('Ctrl Pts',(16.2395131466373,19.7925521223991,-9.86244845694073));
#48634=CARTESIAN_POINT('Ctrl Pts',(16.2599662961795,19.8741854840192,-9.8666140566763));
#48635=CARTESIAN_POINT('Ctrl Pts',(16.2843678510517,19.9545740278134,-9.87077965641186));
#48636=CARTESIAN_POINT('Ctrl Pts',(16.3087969918046,20.035053450603,-9.87494996534479));
#48637=CARTESIAN_POINT('Ctrl Pts',(16.3371833165997,20.1142848040861,-9.87912027427772));
#48638=CARTESIAN_POINT('Ctrl Pts',(16.3693624790257,20.191861557204,-9.88329058321065));
#48639=CARTESIAN_POINT('Ctrl Pts',(16.4015603628986,20.2694834435371,-9.88746331837879));
#48640=CARTESIAN_POINT('Ctrl Pts',(16.437555280145,20.3454483968708,-9.89163605354694));
#48641=CARTESIAN_POINT('Ctrl Pts',(16.4771361744286,20.4193731513184,-9.89580878871509));
#48642=CARTESIAN_POINT('Ctrl Pts',(16.5167895617082,20.4934333000524,-9.8999891663097));
#48643=CARTESIAN_POINT('Ctrl Pts',(16.5600418069655,20.5654453913553,-9.90416954390431));
#48644=CARTESIAN_POINT('Ctrl Pts',(16.6066377495773,20.6350540212634,-9.90834992149893));
#48645=CARTESIAN_POINT('Ctrl Pts',(16.6436006876733,20.6902721225405,-9.91166606942054));
#48646=CARTESIAN_POINT('Ctrl Pts',(16.6826668124624,20.7439783287842,-9.91498221734214));
#48647=CARTESIAN_POINT('Ctrl Pts',(16.7236914224215,20.7960108589263,-9.91829836526375));
#48648=CARTESIAN_POINT('Ctrl Pts',(16.7754602209958,20.8616705099242,-9.9224829996568));
#48649=CARTESIAN_POINT('Ctrl Pts',(16.8305455538229,20.924913415419,-9.92666763404985));
#48650=CARTESIAN_POINT('Ctrl Pts',(16.8886933634204,20.9853853631597,-9.93085226844291));
#48651=CARTESIAN_POINT('Ctrl Pts',(16.9467584068082,21.0457712365676,-9.93503094652685));
#48652=CARTESIAN_POINT('Ctrl Pts',(17.0078769523777,21.1033936577097,-9.9392096246108));
#48653=CARTESIAN_POINT('Ctrl Pts',(17.07175395795,21.157930429083,-9.94338830269474));
#48654=CARTESIAN_POINT('Ctrl Pts',(17.1367759129396,21.2134447328882,-9.94764188058018));
#48655=CARTESIAN_POINT('Ctrl Pts',(17.2046558928942,21.2657612997092,-9.95189545846561));
#48656=CARTESIAN_POINT('Ctrl Pts',(17.2750424589418,21.314578592159,-9.95614903635105));
#48657=CARTESIAN_POINT('Ctrl Pts',(17.3440644440585,21.3624494661354,-9.960320150329));
#48658=CARTESIAN_POINT('Ctrl Pts',(17.4154962970282,21.406955261226,-9.96449126430695));
#48659=CARTESIAN_POINT('Ctrl Pts',(17.4889737195064,21.4478526015096,-9.9686623782849));
#48660=CARTESIAN_POINT('Ctrl Pts',(17.5624264859259,21.4887362182957,-9.97283209260528));
#48661=CARTESIAN_POINT('Ctrl Pts',(17.6379230570028,21.5260135615005,-9.97700180692565));
#48662=CARTESIAN_POINT('Ctrl Pts',(17.7150725574696,21.5594860797668,-9.98117152124602));
#48663=CARTESIAN_POINT('Ctrl Pts',(17.7922193126263,21.5929574069373,-9.98534108719007));
#48664=CARTESIAN_POINT('Ctrl Pts',(17.871018457864,21.6226239960436,-9.98951065313412));
#48665=CARTESIAN_POINT('Ctrl Pts',(17.9510583236147,21.6483350880375,-9.99368021907817));
#48666=CARTESIAN_POINT('Ctrl Pts',(18.0339122923051,21.6749501503078,-9.99799638181709));
#48667=CARTESIAN_POINT('Ctrl Pts',(18.118095350145,21.6973262283485,-10.002312544556));
#48668=CARTESIAN_POINT('Ctrl Pts',(18.2031347548814,21.7153526292288,-10.0066287072949));
#48669=CARTESIAN_POINT('Ctrl Pts',(18.2854040099532,21.7327918219965,-10.0108042714866));
#48670=CARTESIAN_POINT('Ctrl Pts',(18.3684742051326,21.7461603390116,-10.0149798356783));
#48671=CARTESIAN_POINT('Ctrl Pts',(18.4519097174451,21.7554105550182,-10.01915539987));
#48672=CARTESIAN_POINT('Ctrl Pts',(18.5395593591353,21.765127977445,-10.0235418618825));
#48673=CARTESIAN_POINT('Ctrl Pts',(18.6276116092813,21.7703001003685,-10.027928323895));
#48674=CARTESIAN_POINT('Ctrl Pts',(18.7155609817199,21.7709335933975,-10.0323147859076));
#48675=CARTESIAN_POINT('Ctrl Pts',(18.8035103541584,21.7715670864265,-10.0367012479201));
#48676=CARTESIAN_POINT('Ctrl Pts',(18.891356272623,21.767662051318,-10.0410877099327));
#48677=CARTESIAN_POINT('Ctrl Pts',(18.9786013944248,21.7592876913421,-10.0454741719452));
#48678=CARTESIAN_POINT('Ctrl Pts',(19.0618259169023,21.7512992549039,-10.0496584884871));
#48679=CARTESIAN_POINT('Ctrl Pts',(19.14481355195,21.7392146225067,-10.0538428050291));
#48680=CARTESIAN_POINT('Ctrl Pts',(19.2271290458152,21.7230556809461,-10.058027121571));
#48681=CARTESIAN_POINT('Ctrl Pts',(19.3093328037827,21.7069186736988,-10.0622057582787));
#48682=CARTESIAN_POINT('Ctrl Pts',(19.3908657848194,21.6867184269618,-10.0663843949863));
#48683=CARTESIAN_POINT('Ctrl Pts',(19.4712973833544,21.6625286187395,-10.070563031694));
#48684=CARTESIAN_POINT('Ctrl Pts',(19.5516353626659,21.6383669665044,-10.0747368046325));
#48685=CARTESIAN_POINT('Ctrl Pts',(19.6308740694803,21.6102251148652,-10.0789105775711));
#48686=CARTESIAN_POINT('Ctrl Pts',(19.708594110491,21.578227559783,-10.0830843505096));
#48687=CARTESIAN_POINT('Ctrl Pts',(19.786260803981,21.5462519680221,-10.0872552585444));
#48688=CARTESIAN_POINT('Ctrl Pts',(19.8624104781162,21.5104261042933,-10.0914261665791));
#48689=CARTESIAN_POINT('Ctrl Pts',(19.9366409846833,21.4709235964873,-10.0955970746139));
#48690=CARTESIAN_POINT('Ctrl Pts',(20.0108540887569,21.4314303495925,-10.099767004827));
#48691=CARTESIAN_POINT('Ctrl Pts',(20.08314850986,21.3882623802746,-10.1039369350401));
#48692=CARTESIAN_POINT('Ctrl Pts',(20.1531451666036,21.3416400437675,-10.1081068652532));
#48693=CARTESIAN_POINT('Ctrl Pts',(20.2010560876092,21.3097282470417,-10.1109610758159));
#48694=CARTESIAN_POINT('Ctrl Pts',(20.2478909716886,21.276199040298,-10.1138152863787));
#48695=CARTESIAN_POINT('Ctrl Pts',(20.2935358855687,21.2411349269503,-10.1166694969415));
#48696=CARTESIAN_POINT('',(16.1740010233873,19.2132890482674,-9.76670989018929));
#48697=CARTESIAN_POINT('Ctrl Pts',(16.174001023388,19.2132890490549,-9.76670989022851));
#48698=CARTESIAN_POINT('Ctrl Pts',(16.1741079389015,19.3328599270272,-9.77266511192853));
#48699=CARTESIAN_POINT('Ctrl Pts',(16.1825955516607,19.4520702292312,-9.77862033362856));
#48700=CARTESIAN_POINT('Ctrl Pts',(16.1992930219785,19.5699714968759,-9.78457555532858));
#48701=CARTESIAN_POINT('Ctrl Pts',(16.2067339930653,19.6225123852222,-9.78722940837587));
#48702=CARTESIAN_POINT('Ctrl Pts',(16.2158047738395,19.6747937484515,-9.78988326142315));
#48703=CARTESIAN_POINT('Ctrl Pts',(16.2264874578014,19.7267333135613,-9.79253711447044));
#48704=CARTESIAN_POINT('Ctrl Pts',(16.2433320704913,19.8086323813112,-9.79672174886349));
#48705=CARTESIAN_POINT('Ctrl Pts',(16.2642246666771,19.8898577370365,-9.80090638325653));
#48706=CARTESIAN_POINT('Ctrl Pts',(16.2890969179465,19.969978866218,-9.80509101764958));
#48707=CARTESIAN_POINT('Ctrl Pts',(16.3139337666449,20.0499859528891,-9.80926969573353));
#48708=CARTESIAN_POINT('Ctrl Pts',(16.3427388836329,20.1288914993742,-9.81344837381748));
#48709=CARTESIAN_POINT('Ctrl Pts',(16.3753929533288,20.2062752380084,-9.81762705190142));
#48710=CARTESIAN_POINT('Ctrl Pts',(16.4086323237558,20.2850460245429,-9.82188062978686));
#48711=CARTESIAN_POINT('Ctrl Pts',(16.4458598919279,20.3622394375428,-9.82613420767229));
#48712=CARTESIAN_POINT('Ctrl Pts',(16.4868966678982,20.4374283977701,-9.83038778555773));
#48713=CARTESIAN_POINT('Ctrl Pts',(16.5271378658896,20.5111596732842,-9.83455889953568));
#48714=CARTESIAN_POINT('Ctrl Pts',(16.5710416613174,20.5829631005169,-9.83873001351363));
#48715=CARTESIAN_POINT('Ctrl Pts',(16.6183914981669,20.6524578269833,-9.84290112749158));
#48716=CARTESIAN_POINT('Ctrl Pts',(16.6657254463213,20.7219292338231,-9.84707084181195));
#48717=CARTESIAN_POINT('Ctrl Pts',(16.7165028805481,20.7890930986176,-9.85124055613233));
#48718=CARTESIAN_POINT('Ctrl Pts',(16.7704633948897,20.8535967248207,-9.8554102704527));
#48719=CARTESIAN_POINT('Ctrl Pts',(16.8244219890847,20.9180980557081,-9.85957983639674));
#48720=CARTESIAN_POINT('Ctrl Pts',(16.8815631423605,20.9799389839165,-9.86374940234079));
#48721=CARTESIAN_POINT('Ctrl Pts',(16.9415864376591,21.0388002137915,-9.86791896828483));
#48722=CARTESIAN_POINT('Ctrl Pts',(17.0037200779736,21.0997309318957,-9.87223513102375));
#48723=CARTESIAN_POINT('Ctrl Pts',(17.0689419268742,21.1574681514489,-9.87655129376267));
#48724=CARTESIAN_POINT('Ctrl Pts',(17.1368790142891,21.2117010163945,-9.88086745650159));
#48725=CARTESIAN_POINT('Ctrl Pts',(17.2026030582273,21.2641672514687,-9.88504302069327));
#48726=CARTESIAN_POINT('Ctrl Pts',(17.270867749702,21.3133536974898,-9.88921858488495));
#48727=CARTESIAN_POINT('Ctrl Pts',(17.3413050297812,21.3590225138316,-9.89339414907663));
#48728=CARTESIAN_POINT('Ctrl Pts',(17.4152999294285,21.4069979535195,-9.89778061108917));
#48729=CARTESIAN_POINT('Ctrl Pts',(17.4916921547949,21.4510907819032,-9.9021670731017));
#48730=CARTESIAN_POINT('Ctrl Pts',(17.5700268579946,21.4910803768047,-9.90655353511425));
#48731=CARTESIAN_POINT('Ctrl Pts',(17.6483615611942,21.5310699717063,-9.91093999712678));
#48732=CARTESIAN_POINT('Ctrl Pts',(17.7286381814852,21.5669561657755,-9.91532645913933));
#48733=CARTESIAN_POINT('Ctrl Pts',(17.8103811197832,21.5985778865007,-9.91971292115187));
#48734=CARTESIAN_POINT('Ctrl Pts',(17.8883629443181,21.6287446449807,-9.92389755554492));
#48735=CARTESIAN_POINT('Ctrl Pts',(17.9679693803479,21.6551430224068,-9.92808218993796));
#48736=CARTESIAN_POINT('Ctrl Pts',(18.0488014484185,21.6775974428168,-9.93226682433101));
#48737=CARTESIAN_POINT('Ctrl Pts',(18.1295184620453,21.7000199021387,-9.93644550241496));
#48738=CARTESIAN_POINT('Ctrl Pts',(18.2114572030592,21.7185094330108,-9.9406241804989));
#48739=CARTESIAN_POINT('Ctrl Pts',(18.2941997096014,21.7329388780391,-9.94480285858285));
#48740=CARTESIAN_POINT('Ctrl Pts',(18.3784253161073,21.7476269604994,-9.94905643646828));
#48741=CARTESIAN_POINT('Ctrl Pts',(18.4634833368926,21.758107797425,-9.95331001435372));
#48742=CARTESIAN_POINT('Ctrl Pts',(18.5489177820416,21.7643007211442,-9.95756359223915));
#48743=CARTESIAN_POINT('Ctrl Pts',(18.6326959137598,21.7703735829526,-9.96173470621711));
#48744=CARTESIAN_POINT('Ctrl Pts',(18.7168355246875,21.7723232722254,-9.96590582019506));
#48745=CARTESIAN_POINT('Ctrl Pts',(18.8008991604928,21.7701257300737,-9.97007693417301));
#48746=CARTESIAN_POINT('Ctrl Pts',(18.8849345879333,21.7679289253285,-9.97424664849339));
#48747=CARTESIAN_POINT('Ctrl Pts',(18.9688936313901,21.7615876649968,-9.97841636281376));
#48748=CARTESIAN_POINT('Ctrl Pts',(19.0523387760779,21.7511300013277,-9.98258607713413));
#48749=CARTESIAN_POINT('Ctrl Pts',(19.1357809514293,21.7406727097872,-9.98675564307818));
#48750=CARTESIAN_POINT('Ctrl Pts',(19.2187088080141,21.726099364199,-9.99092520902222));
#48751=CARTESIAN_POINT('Ctrl Pts',(19.3006912586606,21.7074897390852,-9.99509477496627));
#48752=CARTESIAN_POINT('Ctrl Pts',(19.3855561111356,21.6882258225098,-9.99941093770518));
#48753=CARTESIAN_POINT('Ctrl Pts',(19.4694073254465,21.6646366310369,-10.0037271004441));
#48754=CARTESIAN_POINT('Ctrl Pts',(19.5517816392177,21.6368675129855,-10.008043263183));
#48755=CARTESIAN_POINT('Ctrl Pts',(19.631472618382,21.6100029710338,-10.0122188273747));
#48756=CARTESIAN_POINT('Ctrl Pts',(19.7097810183149,21.5792268589616,-10.0163943915664));
#48757=CARTESIAN_POINT('Ctrl Pts',(19.7863076293697,21.5447199174645,-10.0205699557581));
#48758=CARTESIAN_POINT('Ctrl Pts',(19.8666994176241,21.5084701123847,-10.0249564177706));
#48759=CARTESIAN_POINT('Ctrl Pts',(19.9451241711511,21.4681029519008,-10.0293428797831));
#48760=CARTESIAN_POINT('Ctrl Pts',(20.0211501810795,21.423881472503,-10.0337293417957));
#48761=CARTESIAN_POINT('Ctrl Pts',(20.0971761910079,21.3796599931052,-10.0381158038082));
#48762=CARTESIAN_POINT('Ctrl Pts',(20.1708030131037,21.3315845757053,-10.0425022658208));
#48763=CARTESIAN_POINT('Ctrl Pts',(20.2416377781111,21.2799679383722,-10.0468887278333));
#48764=CARTESIAN_POINT('Ctrl Pts',(20.2590918809816,21.267249295235,-10.0479695778819));
#48765=CARTESIAN_POINT('Ctrl Pts',(20.2763933923835,21.2543036739806,-10.0490504279306));
#48766=CARTESIAN_POINT('Ctrl Pts',(20.2935358855687,21.2411349269503,-10.0501312779792));
#48767=CARTESIAN_POINT('Ctrl Pts',(20.2935358855687,21.2411349269503,-9.25004024781016));
#48768=CARTESIAN_POINT('Ctrl Pts',(20.3602016680315,21.1899227248892,-9.25421688790189));
#48769=CARTESIAN_POINT('Ctrl Pts',(20.4242843918201,21.1354677868026,-9.25839352799362));
#48770=CARTESIAN_POINT('Ctrl Pts',(20.4854677333106,21.0780727835764,-9.26257016808535));
#48771=CARTESIAN_POINT('Ctrl Pts',(20.546756242997,21.0205791239384,-9.26675398741399));
#48772=CARTESIAN_POINT('Ctrl Pts',(20.6051350976159,20.9601356375273,-9.27093780674262));
#48773=CARTESIAN_POINT('Ctrl Pts',(20.6603262817686,20.8970803824752,-9.27512162607126));
#48774=CARTESIAN_POINT('Ctrl Pts',(20.6986357784777,20.8533122495207,-9.27802571329574));
#48775=CARTESIAN_POINT('Ctrl Pts',(20.7354102689322,20.8082864597362,-9.28092980052022));
#48776=CARTESIAN_POINT('Ctrl Pts',(20.7705691100607,20.7621241923026,-9.28383388774471));
#48777=CARTESIAN_POINT('Ctrl Pts',(20.8212311199913,20.6956068334797,-9.28801852213775));
#48778=CARTESIAN_POINT('Ctrl Pts',(20.8687251499198,20.6264810343216,-9.2922031565308));
#48779=CARTESIAN_POINT('Ctrl Pts',(20.9127716012343,20.5550812139358,-9.29638779092385));
#48780=CARTESIAN_POINT('Ctrl Pts',(20.9567553578771,20.4837830223567,-9.30056646900779));
#48781=CARTESIAN_POINT('Ctrl Pts',(20.9973010436861,20.4102176270062,-9.30474514709174));
#48782=CARTESIAN_POINT('Ctrl Pts',(21.0341702903064,20.3347511448678,-9.30892382517568));
#48783=CARTESIAN_POINT('Ctrl Pts',(21.071700391675,20.2579319802738,-9.31317740306112));
#48784=CARTESIAN_POINT('Ctrl Pts',(21.1054206649962,20.17914328813,-9.31743098094655));
#48785=CARTESIAN_POINT('Ctrl Pts',(21.1351268232138,20.0988006413847,-9.32168455883199));
#48786=CARTESIAN_POINT('Ctrl Pts',(21.1642570695877,20.0200155936222,-9.32585567280994));
#48787=CARTESIAN_POINT('Ctrl Pts',(21.1895272879509,19.939736757811,-9.33002678678789));
#48788=CARTESIAN_POINT('Ctrl Pts',(21.2107927216344,19.8583776440833,-9.33419790076585));
#48789=CARTESIAN_POINT('Ctrl Pts',(21.2320510194963,19.7770458311919,-9.33836761508622));
#48790=CARTESIAN_POINT('Ctrl Pts',(21.2493070853372,19.6946349050202,-9.34253732940659));
#48791=CARTESIAN_POINT('Ctrl Pts',(21.2624662014641,19.6115729247637,-9.34670704372696));
#48792=CARTESIAN_POINT('Ctrl Pts',(21.2756248493332,19.5285139002089,-9.350876609671));
#48793=CARTESIAN_POINT('Ctrl Pts',(21.284686766209,19.4448043221314,-9.35504617561505));
#48794=CARTESIAN_POINT('Ctrl Pts',(21.2896087040397,19.3608804584878,-9.35921574155909));
#48795=CARTESIAN_POINT('Ctrl Pts',(21.2947036911327,19.2740059353297,-9.36353190429801));
#48796=CARTESIAN_POINT('Ctrl Pts',(21.2953621283496,19.1869023041988,-9.36784806703693));
#48797=CARTESIAN_POINT('Ctrl Pts',(21.2915948078576,19.1000549738832,-9.37216422977585));
#48798=CARTESIAN_POINT('Ctrl Pts',(21.2879502074343,19.0160366862179,-9.37633979396754));
#48799=CARTESIAN_POINT('Ctrl Pts',(21.2801638500694,18.9322587224487,-9.38051535815921));
#48800=CARTESIAN_POINT('Ctrl Pts',(21.2682983360669,18.8491548068461,-9.38469092235089));
#48801=CARTESIAN_POINT('Ctrl Pts',(21.2558335231597,18.7618535100273,-9.38907738436343));
#48802=CARTESIAN_POINT('Ctrl Pts',(21.2388667599596,18.675296716199,-9.39346384637597));
#48803=CARTESIAN_POINT('Ctrl Pts',(21.2175306593405,18.5899722517346,-9.39785030838851));
#48804=CARTESIAN_POINT('Ctrl Pts',(21.1961945587214,18.5046477872701,-9.40223677040106));
#48805=CARTESIAN_POINT('Ctrl Pts',(21.1704893630394,18.4205561848055,-9.4066232324136));
#48806=CARTESIAN_POINT('Ctrl Pts',(21.1406062076889,18.3381617783842,-9.41100969442614));
#48807=CARTESIAN_POINT('Ctrl Pts',(21.1120980206135,18.2595584607401,-9.41519432881919));
#48808=CARTESIAN_POINT('Ctrl Pts',(21.0796817805212,18.1822070136536,-9.41937896321224));
#48809=CARTESIAN_POINT('Ctrl Pts',(21.0434873395327,18.1065235500301,-9.42356359760529));
#48810=CARTESIAN_POINT('Ctrl Pts',(21.007344416851,18.0309478124492,-9.42774227568923));
#48811=CARTESIAN_POINT('Ctrl Pts',(20.967434172056,17.9570357539526,-9.43192095377318));
#48812=CARTESIAN_POINT('Ctrl Pts',(20.9239354273224,17.8851859767831,-9.43609963185712));
#48813=CARTESIAN_POINT('Ctrl Pts',(20.8796569988514,17.8120483439955,-9.44035320974256));
#48814=CARTESIAN_POINT('Ctrl Pts',(20.8316603217325,17.7410481057697,-9.44460678762799));
#48815=CARTESIAN_POINT('Ctrl Pts',(20.7801842503405,17.6725819769456,-9.44886036551343));
#48816=CARTESIAN_POINT('Ctrl Pts',(20.7297061430397,17.6054431976295,-9.45303147949138));
#48817=CARTESIAN_POINT('Ctrl Pts',(20.6758826364361,17.5407415318687,-9.45720259346933));
#48818=CARTESIAN_POINT('Ctrl Pts',(20.618983073072,17.4788225223055,-9.46137370744728));
#48819=CARTESIAN_POINT('Ctrl Pts',(20.5621026029059,17.416924290264,-9.46554342176766));
#48820=CARTESIAN_POINT('Ctrl Pts',(20.5021484369599,17.3578071984335,-9.46971313608803));
#48821=CARTESIAN_POINT('Ctrl Pts',(20.4394292363846,17.3017825897283,-9.4738828504084));
#48822=CARTESIAN_POINT('Ctrl Pts',(20.3767122676277,17.2457599746191,-9.47805241635244));
#48823=CARTESIAN_POINT('Ctrl Pts',(20.3112308035245,17.1928299296704,-9.48222198229649));
#48824=CARTESIAN_POINT('Ctrl Pts',(20.2433282670354,17.1432649632199,-9.48639154824053));
#48825=CARTESIAN_POINT('Ctrl Pts',(20.1730383611302,17.0919573536941,-9.49070771097945));
#48826=CARTESIAN_POINT('Ctrl Pts',(20.1001543913748,17.0442561687145,-9.49502387371837));
#48827=CARTESIAN_POINT('Ctrl Pts',(20.025090351338,17.000415076347,-9.49934003645729));
#48828=CARTESIAN_POINT('Ctrl Pts',(19.9524715145099,16.9580021029521,-9.50351560064897));
#48829=CARTESIAN_POINT('Ctrl Pts',(19.8778128975685,16.9192017744647,-9.50769116484065));
#48830=CARTESIAN_POINT('Ctrl Pts',(19.8015130783443,16.8841962206572,-9.51186672903234));
#48831=CARTESIAN_POINT('Ctrl Pts',(19.7213595366366,16.8474226195447,-9.51625319104488));
#48832=CARTESIAN_POINT('Ctrl Pts',(19.6393951838166,16.8148374315278,-9.52063965305742));
#48833=CARTESIAN_POINT('Ctrl Pts',(19.5561019854973,16.7865932013292,-9.52502611506996));
#48834=CARTESIAN_POINT('Ctrl Pts',(19.472808787178,16.7583489711306,-9.5294125770825));
#48835=CARTESIAN_POINT('Ctrl Pts',(19.3881873224049,16.7344457832731,-9.53379903909503));
#48836=CARTESIAN_POINT('Ctrl Pts',(19.3027314805897,16.7149742583486,-9.53818550110757));
#48837=CARTESIAN_POINT('Ctrl Pts',(19.2212075887324,16.6963986471497,-9.54237013550062));
#48838=CARTESIAN_POINT('Ctrl Pts',(19.1386209669252,16.6817867038644,-9.54655476989367));
#48839=CARTESIAN_POINT('Ctrl Pts',(19.0553917867604,16.6712544774322,-9.55073940428672));
#48840=CARTESIAN_POINT('Ctrl Pts',(18.9722810730319,16.6607372423208,-9.55491808237066));
#48841=CARTESIAN_POINT('Ctrl Pts',(18.8885300701232,16.654288246849,-9.5590967604546));
#48842=CARTESIAN_POINT('Ctrl Pts',(18.8045707324921,16.6519728857014,-9.56327543853854));
#48843=CARTESIAN_POINT('Ctrl Pts',(18.7191064840744,16.6496160233692,-9.56752901642398));
#48844=CARTESIAN_POINT('Ctrl Pts',(18.6334268287623,16.6515425508617,-9.57178259430941));
#48845=CARTESIAN_POINT('Ctrl Pts',(18.5479946282975,16.6577663636679,-9.57603617219485));
#48846=CARTESIAN_POINT('Ctrl Pts',(18.464218697746,16.663869515718,-9.5802072861728));
#48847=CARTESIAN_POINT('Ctrl Pts',(18.3806811928208,16.6741047825048,-9.58437840015076));
#48848=CARTESIAN_POINT('Ctrl Pts',(18.2978184502104,16.6884327252533,-9.58854951412871));
#48849=CARTESIAN_POINT('Ctrl Pts',(18.2149835129936,16.7027558601221,-9.59271922844908));
#48850=CARTESIAN_POINT('Ctrl Pts',(18.1328233413408,16.7211688651668,-9.59688894276946));
#48851=CARTESIAN_POINT('Ctrl Pts',(18.0517667977986,16.7435807292205,-9.60105865708983));
#48852=CARTESIAN_POINT('Ctrl Pts',(17.970713138596,16.7659917957639,-9.60522822303387));
#48853=CARTESIAN_POINT('Ctrl Pts',(17.8907634725905,16.7924013149753,-9.60939778897792));
#48854=CARTESIAN_POINT('Ctrl Pts',(17.8123328245036,16.8226680260876,-9.61356735492196));
#48855=CARTESIAN_POINT('Ctrl Pts',(17.7311446515846,16.8539988774245,-9.61788351766088));
#48856=CARTESIAN_POINT('Ctrl Pts',(17.6515847934182,16.8894630151456,-9.6221996803998));
#48857=CARTESIAN_POINT('Ctrl Pts',(17.5740906315705,16.9288496418883,-9.62651584313872));
#48858=CARTESIAN_POINT('Ctrl Pts',(17.4991208338941,16.9669532534076,-9.6306914073304));
#48859=CARTESIAN_POINT('Ctrl Pts',(17.4260846045836,17.0087274533692,-9.63486697152208));
#48860=CARTESIAN_POINT('Ctrl Pts',(17.3553508285749,17.0539356842855,-9.63904253571376));
#48861=CARTESIAN_POINT('Ctrl Pts',(17.2810444576937,17.101427275473,-9.64342899772631));
#48862=CARTESIAN_POINT('Ctrl Pts',(17.2092797216846,17.1527085808079,-9.64781545973885));
#48863=CARTESIAN_POINT('Ctrl Pts',(17.1404457653641,17.2074569130478,-9.65220192175139));
#48864=CARTESIAN_POINT('Ctrl Pts',(17.0716118090436,17.2622052452876,-9.65658838376393));
#48865=CARTESIAN_POINT('Ctrl Pts',(17.0057090169082,17.3204201632973,-9.66097484577647));
#48866=CARTESIAN_POINT('Ctrl Pts',(16.9430809195061,17.3817354354488,-9.66536130778901));
#48867=CARTESIAN_POINT('Ctrl Pts',(16.8827886985013,17.4407637964061,-9.66958416538902));
#48868=CARTESIAN_POINT('Ctrl Pts',(16.8252872091303,17.5029045422553,-9.67380702298903));
#48869=CARTESIAN_POINT('Ctrl Pts',(16.7709203169311,17.5678572314245,-9.67802988058904));
#48870=CARTESIAN_POINT('Ctrl Pts',(16.7179063153622,17.6311936081462,-9.68214765466764));
#48871=CARTESIAN_POINT('Ctrl Pts',(16.6678730797622,17.6972032456021,-9.68626542874624));
#48872=CARTESIAN_POINT('Ctrl Pts',(16.6211045875939,17.7655682388182,-9.69038320282484));
#48873=CARTESIAN_POINT('Ctrl Pts',(16.57438033231,17.833868567681,-9.69449708202705));
#48874=CARTESIAN_POINT('Ctrl Pts',(16.530914960773,17.9045194435154,-9.69861096122926));
#48875=CARTESIAN_POINT('Ctrl Pts',(16.4909521572678,17.9771700379653,-9.70272484043147));
#48876=CARTESIAN_POINT('Ctrl Pts',(16.451014356568,18.0497751784301,-9.70683614577719));
#48877=CARTESIAN_POINT('Ctrl Pts',(16.4145750025456,18.1243771397533,-9.7109474511229));
#48878=CARTESIAN_POINT('Ctrl Pts',(16.3818335581791,18.2005975900802,-9.71505875646862));
#48879=CARTESIAN_POINT('Ctrl Pts',(16.3475554603697,18.2803952930204,-9.71936301761201));
#48880=CARTESIAN_POINT('Ctrl Pts',(16.3173311789841,18.3619666588744,-9.7236672787554));
#48881=CARTESIAN_POINT('Ctrl Pts',(16.2913340385439,18.4448518415191,-9.72797153989879));
#48882=CARTESIAN_POINT('Ctrl Pts',(16.2665001036005,18.5240284432035,-9.73208321292914));
#48883=CARTESIAN_POINT('Ctrl Pts',(16.2455232446819,18.6044033134949,-9.73619488595948));
#48884=CARTESIAN_POINT('Ctrl Pts',(16.2285034541843,18.685560128173,-9.74030655898983));
#48885=CARTESIAN_POINT('Ctrl Pts',(16.2114791195103,18.7667386112068,-9.74441932981085));
#48886=CARTESIAN_POINT('Ctrl Pts',(16.1984140354435,18.84869898642,-9.74853210063186));
#48887=CARTESIAN_POINT('Ctrl Pts',(16.1893567554131,18.9310165044539,-9.75264487145288));
#48888=CARTESIAN_POINT('Ctrl Pts',(16.1802905487374,19.0134151527258,-9.7567616957255));
#48889=CARTESIAN_POINT('Ctrl Pts',(16.1752400549859,19.0961711731434,-9.76087851999813));
#48890=CARTESIAN_POINT('Ctrl Pts',(16.1742017924823,19.1788575547115,-9.76499534427075));
#48891=CARTESIAN_POINT('Ctrl Pts',(16.1740576564023,19.1903364349233,-9.76556685957693));
#48892=CARTESIAN_POINT('Ctrl Pts',(16.1739907628404,19.2018139780891,-9.76613837488311));
#48893=CARTESIAN_POINT('Ctrl Pts',(16.1740010233873,19.2132890482674,-9.76670989018929));
#48894=CARTESIAN_POINT('Origin',(18.734,19.211,1.76670989022852));
#48895=CARTESIAN_POINT('',(20.2935358855687,21.2411349269503,-8.45013430427981));
#48896=CARTESIAN_POINT('',(20.2935358855687,21.2411349269503,-8.51667715193081));
#48897=CARTESIAN_POINT('',(20.2935358855687,21.2411349269503,1.76670989022852));
#48898=CARTESIAN_POINT('',(16.1736699135442,19.2103574886798,-9.03329016588334));
#48899=CARTESIAN_POINT('Ctrl Pts',(20.2935358855687,21.2411349269503,-8.51667715193082));
#48900=CARTESIAN_POINT('Ctrl Pts',(20.3077409106736,21.2302227229818,-8.51757293187653));
#48901=CARTESIAN_POINT('Ctrl Pts',(20.3218260012755,21.2191655684692,-8.51846871182225));
#48902=CARTESIAN_POINT('Ctrl Pts',(20.3357880909557,21.2079664272773,-8.51936449176796));
#48903=CARTESIAN_POINT('Ctrl Pts',(20.4010119675942,21.1556496594946,-8.52354912616101));
#48904=CARTESIAN_POINT('Ctrl Pts',(20.463791413314,21.1000367097147,-8.52773376055406));
#48905=CARTESIAN_POINT('Ctrl Pts',(20.5237743555653,21.0413845924179,-8.53191839494711));
#48906=CARTESIAN_POINT('Ctrl Pts',(20.5836719195227,20.9828159591504,-8.53609707303105));
#48907=CARTESIAN_POINT('Ctrl Pts',(20.6407805603834,20.9212170697946,-8.540275751115));
#48908=CARTESIAN_POINT('Ctrl Pts',(20.6947805623983,20.8568856540237,-8.54445442919895));
#48909=CARTESIAN_POINT('Ctrl Pts',(20.7497484756403,20.7914011438593,-8.54870800708438));
#48910=CARTESIAN_POINT('Ctrl Pts',(20.8014948330691,20.7230854843409,-8.55296158496981));
#48911=CARTESIAN_POINT('Ctrl Pts',(20.8497210505506,20.6522926268656,-8.55721516285525));
#48912=CARTESIAN_POINT('Ctrl Pts',(20.8970123087005,20.5828722270732,-8.5613862768332));
#48913=CARTESIAN_POINT('Ctrl Pts',(20.9409184275291,20.5110702205223,-8.56555739081116));
#48914=CARTESIAN_POINT('Ctrl Pts',(20.9811990900047,20.4372529306314,-8.56972850478911));
#48915=CARTESIAN_POINT('Ctrl Pts',(21.021466235915,20.363460410845,-8.57389821910948));
#48916=CARTESIAN_POINT('Ctrl Pts',(21.058110121399,20.2876543542438,-8.57806793342985));
#48917=CARTESIAN_POINT('Ctrl Pts',(21.0909354749524,20.210227284911,-8.58223764775023));
#48918=CARTESIAN_POINT('Ctrl Pts',(21.123759660439,20.1328029707657,-8.58640721369427));
#48919=CARTESIAN_POINT('Ctrl Pts',(21.1527654053819,20.0537581824512,-8.59057677963832));
#48920=CARTESIAN_POINT('Ctrl Pts',(21.1778054030264,19.9735058374459,-8.59474634558236));
#48921=CARTESIAN_POINT('Ctrl Pts',(21.2037257760978,19.8904319189921,-8.59906250832128));
#48922=CARTESIAN_POINT('Ctrl Pts',(21.2253961847597,19.8060644520147,-8.6033786710602));
#48923=CARTESIAN_POINT('Ctrl Pts',(21.2427098983461,19.7208770890524,-8.60769483379912));
#48924=CARTESIAN_POINT('Ctrl Pts',(21.2594596195334,19.6384646954784,-8.6118703979908));
#48925=CARTESIAN_POINT('Ctrl Pts',(21.2721321012068,19.5552854746202,-8.61604596218248));
#48926=CARTESIAN_POINT('Ctrl Pts',(21.2806833673555,19.4717754329589,-8.62022152637416));
#48927=CARTESIAN_POINT('Ctrl Pts',(21.2896665376286,19.3840474976196,-8.6246079883867));
#48928=CARTESIAN_POINT('Ctrl Pts',(21.2941011966021,19.2959550268227,-8.62899445039924));
#48929=CARTESIAN_POINT('Ctrl Pts',(21.2939982462078,19.2080034331647,-8.63338091241178));
#48930=CARTESIAN_POINT('Ctrl Pts',(21.2938952958136,19.1200518395066,-8.63776737442432));
#48931=CARTESIAN_POINT('Ctrl Pts',(21.2892548426303,19.0322416983818,-8.64215383643686));
#48932=CARTESIAN_POINT('Ctrl Pts',(21.2801502518719,18.9450697555886,-8.6465402984494));
#48933=CARTESIAN_POINT('Ctrl Pts',(21.2714645768305,18.8619087231031,-8.65072493284245));
#48934=CARTESIAN_POINT('Ctrl Pts',(21.2586842102674,18.7790189093826,-8.65490956723549));
#48935=CARTESIAN_POINT('Ctrl Pts',(21.2418346904937,18.6968354687883,-8.65909420162854));
#48936=CARTESIAN_POINT('Ctrl Pts',(21.2250091539259,18.6147690061494,-8.66327287971249));
#48937=CARTESIAN_POINT('Ctrl Pts',(21.2041260603601,18.533407366331,-8.66745155779643));
#48938=CARTESIAN_POINT('Ctrl Pts',(21.1792626972637,18.4531805351071,-8.67163023588037));
#48939=CARTESIAN_POINT('Ctrl Pts',(21.1539536762528,18.3715156955914,-8.67588381376581));
#48940=CARTESIAN_POINT('Ctrl Pts',(21.1245203396143,18.2910272272441,-8.68013739165124));
#48941=CARTESIAN_POINT('Ctrl Pts',(21.0910986865303,18.2121577792478,-8.68439096953668));
#48942=CARTESIAN_POINT('Ctrl Pts',(21.0583249774083,18.1348173694021,-8.68856208351463));
#48943=CARTESIAN_POINT('Ctrl Pts',(21.0217164021894,18.0590342074479,-8.69273319749258));
#48944=CARTESIAN_POINT('Ctrl Pts',(20.9814509018453,17.9852086458966,-8.69690431147054));
#48945=CARTESIAN_POINT('Ctrl Pts',(20.9411989129789,17.9114078572255,-8.70107402579091));
#48946=CARTESIAN_POINT('Ctrl Pts',(20.897292656152,17.8395637678915,-8.70524374011128));
#48947=CARTESIAN_POINT('Ctrl Pts',(20.849956485239,17.7700530361685,-8.70941345443166));
#48948=CARTESIAN_POINT('Ctrl Pts',(20.80262199875,17.7005447779357,-8.7135830203757));
#48949=CARTESIAN_POINT('Ctrl Pts',(20.7518581004866,17.6333700919857,-8.71775258631974));
#48950=CARTESIAN_POINT('Ctrl Pts',(20.6979322543499,17.5688763443869,-8.72192215226378));
#48951=CARTESIAN_POINT('Ctrl Pts',(20.6421104419877,17.5021150761842,-8.7262383150027));
#48952=CARTESIAN_POINT('Ctrl Pts',(20.5829005348977,17.4382271821969,-8.73055447774163));
#48953=CARTESIAN_POINT('Ctrl Pts',(20.5206430286226,17.3775587851599,-8.73487064048055));
#48954=CARTESIAN_POINT('Ctrl Pts',(20.460413554066,17.3188666547752,-8.73904620467223));
#48955=CARTESIAN_POINT('Ctrl Pts',(20.3973323666986,17.2631877685198,-8.74322176886391));
#48956=CARTESIAN_POINT('Ctrl Pts',(20.3317422755907,17.2107951052979,-8.74739733305559));
#48957=CARTESIAN_POINT('Ctrl Pts',(20.2628393849066,17.1557562132084,-8.75178379506813));
#48958=CARTESIAN_POINT('Ctrl Pts',(20.1911679546945,17.1043445831752,-8.75617025708067));
#48959=CARTESIAN_POINT('Ctrl Pts',(20.1171588579738,17.0568246186513,-8.76055671909321));
#48960=CARTESIAN_POINT('Ctrl Pts',(20.043149761253,17.0093046541274,-8.76494318110575));
#48961=CARTESIAN_POINT('Ctrl Pts',(19.9668035395282,16.9656765769471,-8.76932964311829));
#48962=CARTESIAN_POINT('Ctrl Pts',(19.8885775886028,16.9261475776549,-8.77371610513083));
#48963=CARTESIAN_POINT('Ctrl Pts',(19.8139509296381,16.8884373662162,-8.77790073952388));
#48964=CARTESIAN_POINT('Ctrl Pts',(19.7373359438749,16.8543169479217,-8.78208537391693));
#48965=CARTESIAN_POINT('Ctrl Pts',(19.6591123506695,16.8240003898955,-8.78627000830997));
#48966=CARTESIAN_POINT('Ctrl Pts',(19.5810000990668,16.7937269837373,-8.79044868639392));
#48967=CARTESIAN_POINT('Ctrl Pts',(19.5012842132702,16.7672468481168,-8.79462736447787));
#48968=CARTESIAN_POINT('Ctrl Pts',(19.420368077509,16.7447277396491,-8.79880604256181));
#48969=CARTESIAN_POINT('Ctrl Pts',(19.3380015781677,16.7218049923462,-8.80305962044725));
#48970=CARTESIAN_POINT('Ctrl Pts',(19.2543918069889,16.7029868892007,-8.80731319833268));
#48971=CARTESIAN_POINT('Ctrl Pts',(19.1699845756622,16.6883986740302,-8.81156677621811));
#48972=CARTESIAN_POINT('Ctrl Pts',(19.0872137432219,16.6740932798773,-8.81573789019606));
#48973=CARTESIAN_POINT('Ctrl Pts',(19.0036765695344,16.6638553099793,-8.81990900417402));
#48974=CARTESIAN_POINT('Ctrl Pts',(18.9198060037776,16.6577518473599,-8.82408011815197));
#48975=CARTESIAN_POINT('Ctrl Pts',(18.8359635815991,16.6516504328162,-8.82824983247234));
#48976=CARTESIAN_POINT('Ctrl Pts',(18.7517884479705,16.6496808035662,-8.83241954679272));
#48977=CARTESIAN_POINT('Ctrl Pts',(18.6677187513895,16.6518581914863,-8.83658926111309));
#48978=CARTESIAN_POINT('Ctrl Pts',(18.5836520463691,16.6540355019256,-8.84075882705714));
#48979=CARTESIAN_POINT('Ctrl Pts',(18.4996912307931,16.660359523368,-8.84492839300118));
#48980=CARTESIAN_POINT('Ctrl Pts',(18.4162731576902,16.6707933836643,-8.84909795894523));
#48981=CARTESIAN_POINT('Ctrl Pts',(18.3299222080443,16.681594085617,-8.85341412168415));
#48982=CARTESIAN_POINT('Ctrl Pts',(18.2441533999762,16.6967989420232,-8.85773028442307));
#48983=CARTESIAN_POINT('Ctrl Pts',(18.1594420717103,16.7163089996876,-8.86204644716199));
#48984=CARTESIAN_POINT('Ctrl Pts',(18.0774902060527,16.7351835192758,-8.86622201135367));
#48985=CARTESIAN_POINT('Ctrl Pts',(17.996528423794,16.758086889941,-8.87039757554535));
#48986=CARTESIAN_POINT('Ctrl Pts',(17.9169718130409,16.7848786218092,-8.87457313973703));
#48987=CARTESIAN_POINT('Ctrl Pts',(17.8333969870066,16.8130235403628,-8.87895960174957));
#48988=CARTESIAN_POINT('Ctrl Pts',(17.7513735563979,16.8454597306831,-8.88334606376211));
#48989=CARTESIAN_POINT('Ctrl Pts',(17.6713570660694,16.8819680133224,-8.88773252577465));
#48990=CARTESIAN_POINT('Ctrl Pts',(17.5913405757408,16.9184762959617,-8.89211898778719));
#48991=CARTESIAN_POINT('Ctrl Pts',(17.513331505326,16.959056335675,-8.89650544979973));
#48992=CARTESIAN_POINT('Ctrl Pts',(17.4377516489576,17.003435683288,-8.90089191181227));
#48993=CARTESIAN_POINT('Ctrl Pts',(17.365649333817,17.0457730713314,-8.90507654620532));
#48994=CARTESIAN_POINT('Ctrl Pts',(17.2954892230291,17.091725414496,-8.90926118059837));
#48995=CARTESIAN_POINT('Ctrl Pts',(17.2276568480541,17.1410892993693,-8.91344581499142));
#48996=CARTESIAN_POINT('Ctrl Pts',(17.159921024069,17.1903829208624,-8.91762449307535));
#48997=CARTESIAN_POINT('Ctrl Pts',(17.0945067235342,17.2430781703289,-8.92180317115929));
#48998=CARTESIAN_POINT('Ctrl Pts',(17.0317733474474,17.2989266689429,-8.92598184924323));
#48999=CARTESIAN_POINT('Ctrl Pts',(16.9679155206799,17.3557762117571,-8.93023542712867));
#49000=CARTESIAN_POINT('Ctrl Pts',(16.9068360906096,17.4158929154663,-8.9344890050141));
#49001=CARTESIAN_POINT('Ctrl Pts',(16.8488816768788,17.4789697150936,-8.93874258289954));
#49002=CARTESIAN_POINT('Ctrl Pts',(16.792050822547,17.540823647876,-8.94291369687749));
#49003=CARTESIAN_POINT('Ctrl Pts',(16.7382252223475,17.6055235719755,-8.94708481085544));
#49004=CARTESIAN_POINT('Ctrl Pts',(16.6876956296653,17.6727417564176,-8.9512559248334));
#49005=CARTESIAN_POINT('Ctrl Pts',(16.637182992676,17.7399373851488,-8.95542563915377));
#49006=CARTESIAN_POINT('Ctrl Pts',(16.5899644428518,17.8096492285707,-8.95959535347414));
#49007=CARTESIAN_POINT('Ctrl Pts',(16.5462899492621,17.8815171178611,-8.96376506779451));
#49008=CARTESIAN_POINT('Ctrl Pts',(16.5026170097983,17.9533824497836,-8.96793463373855));
#49009=CARTESIAN_POINT('Ctrl Pts',(16.4624881140049,18.0274032814579,-8.9721041996826));
#49010=CARTESIAN_POINT('Ctrl Pts',(16.4261087184981,18.1031923304257,-8.97627376562664));
#49011=CARTESIAN_POINT('Ctrl Pts',(16.3884502683242,18.1816460288594,-8.98058992836556));
#49012=CARTESIAN_POINT('Ctrl Pts',(16.3548101172679,18.2619941236263,-8.98490609110448));
#49013=CARTESIAN_POINT('Ctrl Pts',(16.3253623529172,18.3437833690158,-8.9892222538434));
#49014=CARTESIAN_POINT('Ctrl Pts',(16.296873846393,18.4229083383394,-8.99339781803508));
#49015=CARTESIAN_POINT('Ctrl Pts',(16.2723088794104,18.5033815448835,-8.99757338222676));
#49016=CARTESIAN_POINT('Ctrl Pts',(16.2517740015379,18.5847779207351,-9.00174894641844));
#49017=CARTESIAN_POINT('Ctrl Pts',(16.2302019558011,18.6702854340295,-9.00613540843099));
#49018=CARTESIAN_POINT('Ctrl Pts',(16.213077931431,18.7568112533014,-9.01052187044352));
#49019=CARTESIAN_POINT('Ctrl Pts',(16.2004642109876,18.8438536997419,-9.01490833245606));
#49020=CARTESIAN_POINT('Ctrl Pts',(16.1878504905441,18.9308961461825,-9.01929479446861));
#49021=CARTESIAN_POINT('Ctrl Pts',(16.179747051756,19.0184546350337,-9.02368125648115));
#49022=CARTESIAN_POINT('Ctrl Pts',(16.1761531171477,19.10602703261,-9.02806771849369));
#49023=CARTESIAN_POINT('Ctrl Pts',(16.1747268399112,19.1407807303868,-9.0298085155863));
#49024=CARTESIAN_POINT('Ctrl Pts',(16.1740088273484,19.1755636940745,-9.0315493126789));
#49025=CARTESIAN_POINT('Ctrl Pts',(16.1740000808904,19.2103564484228,-9.0332901097715));
#49026=CARTESIAN_POINT('Ctrl Pts',(16.1699656655267,19.2103691596404,-9.03329079541918));
#49027=CARTESIAN_POINT('Ctrl Pts',(16.1727141287504,20.0241270866321,-9.07394170533784));
#49028=CARTESIAN_POINT('Ctrl Pts',(17.0319371680896,21.691475877328,-9.15698455081697));
#49029=CARTESIAN_POINT('Ctrl Pts',(19.1726622419323,21.9356231677813,-9.25149015768804));
#49030=CARTESIAN_POINT('Ctrl Pts',(20.1114245040166,21.382657416907,-9.30534485464049));
#49031=CARTESIAN_POINT('Ctrl Pts',(20.2929505577765,21.2403915309053,-9.31680761603245));
#49032=CARTESIAN_POINT('',(16.174000001606,19.2110906788005,-8.96670989026365));
#49033=CARTESIAN_POINT('Ctrl Pts',(16.174000001606,19.2110906788005,-8.96670989026365));
#49034=CARTESIAN_POINT('Ctrl Pts',(16.1740031377284,19.2996281672636,-8.97108917708311));
#49035=CARTESIAN_POINT('Ctrl Pts',(16.1786036643305,19.388071802769,-8.97546846390256));
#49036=CARTESIAN_POINT('Ctrl Pts',(16.1877467776184,19.4759424985001,-8.97984775072202));
#49037=CARTESIAN_POINT('Ctrl Pts',(16.1969159526896,19.5640636632955,-8.98423952038188));
#49038=CARTESIAN_POINT('Ctrl Pts',(16.2106535575187,19.6516082364872,-8.98863129004175));
#49039=CARTESIAN_POINT('Ctrl Pts',(16.2288531973791,19.7381048257399,-8.99302305970162));
#49040=CARTESIAN_POINT('Ctrl Pts',(16.2470794228643,19.8247277672657,-8.99742124475987));
#49041=CARTESIAN_POINT('Ctrl Pts',(16.2697805833341,19.9102992971043,-9.00181942981813));
#49042=CARTESIAN_POINT('Ctrl Pts',(16.2968004138021,19.9943633748375,-9.00621761487638));
#49043=CARTESIAN_POINT('Ctrl Pts',(16.3238953969119,20.0786612674176,-9.01062803299533));
#49044=CARTESIAN_POINT('Ctrl Pts',(16.3553329301083,20.1614429605719,-9.01503845111429));
#49045=CARTESIAN_POINT('Ctrl Pts',(16.3909082116845,20.2422714829415,-9.01944886923325));
#49046=CARTESIAN_POINT('Ctrl Pts',(16.4178853374884,20.3035646370615,-9.02279333761611));
#49047=CARTESIAN_POINT('Ctrl Pts',(16.4472408225494,20.363735085321,-9.02613780599897));
#49048=CARTESIAN_POINT('Ctrl Pts',(16.478868382946,20.422602818486,-9.02948227438183));
#49049=CARTESIAN_POINT('Ctrl Pts',(16.5184411227219,20.4962587519986,-9.03366690877488));
#49050=CARTESIAN_POINT('Ctrl Pts',(16.5616998679758,20.5681109610611,-9.03785154316793));
#49051=CARTESIAN_POINT('Ctrl Pts',(16.6084559713663,20.6377664778581,-9.04203617756098));
#49052=CARTESIAN_POINT('Ctrl Pts',(16.6551455232309,20.7073228486487,-9.04621485564492));
#49053=CARTESIAN_POINT('Ctrl Pts',(16.7053222910481,20.7746883591286,-9.05039353372887));
#49054=CARTESIAN_POINT('Ctrl Pts',(16.7587517035101,20.8394944480144,-9.05457221181282));
#49055=CARTESIAN_POINT('Ctrl Pts',(16.8131387997914,20.9054621394682,-9.05882578969825));
#49056=CARTESIAN_POINT('Ctrl Pts',(16.8708960667842,20.9687773268414,-9.06307936758369));
#49057=CARTESIAN_POINT('Ctrl Pts',(16.9317298045576,21.0290819955712,-9.06733294546912));
#49058=CARTESIAN_POINT('Ctrl Pts',(16.9913841616171,21.0882175406228,-9.07150405944708));
#49059=CARTESIAN_POINT('Ctrl Pts',(17.0539964254171,21.1444579161298,-9.07567517342503));
#49060=CARTESIAN_POINT('Ctrl Pts',(17.1192501263854,21.1975001499274,-9.07984628740298));
#49061=CARTESIAN_POINT('Ctrl Pts',(17.1844819308442,21.2505245848913,-9.08401600172335));
#49062=CARTESIAN_POINT('Ctrl Pts',(17.2523530554692,21.3003527195435,-9.08818571604372));
#49063=CARTESIAN_POINT('Ctrl Pts',(17.3225130695873,21.3467211066228,-9.0923554303641));
#49064=CARTESIAN_POINT('Ctrl Pts',(17.392670587111,21.3930878437159,-9.09652499630815));
#49065=CARTESIAN_POINT('Ctrl Pts',(17.4651164479275,21.4359948250818,-9.10069456225219));
#49066=CARTESIAN_POINT('Ctrl Pts',(17.5394714392698,21.475222055718,-9.10486412819624));
#49067=CARTESIAN_POINT('Ctrl Pts',(17.6164406603809,21.5158284673913,-9.10918029093516));
#49068=CARTESIAN_POINT('Ctrl Pts',(17.6954552934395,21.5524913076844,-9.11349645367408));
#49069=CARTESIAN_POINT('Ctrl Pts',(17.7760690203245,21.585019426664,-9.117812616413));
#49070=CARTESIAN_POINT('Ctrl Pts',(17.8540567635352,21.6164879455891,-9.12198818060468));
#49071=CARTESIAN_POINT('Ctrl Pts',(17.9335405590285,21.6440868736177,-9.12616374479636));
#49072=CARTESIAN_POINT('Ctrl Pts',(18.0140996850997,21.6676936187906,-9.13033930898804));
#49073=CARTESIAN_POINT('Ctrl Pts',(18.0987276611176,21.6924926845425,-9.13472577100058));
#49074=CARTESIAN_POINT('Ctrl Pts',(18.1845418843916,21.7128855434687,-9.13911223301312));
#49075=CARTESIAN_POINT('Ctrl Pts',(18.2710433987723,21.7287909336122,-9.14349869502566));
#49076=CARTESIAN_POINT('Ctrl Pts',(18.3575449131529,21.7446963237556,-9.1478851570382));
#49077=CARTESIAN_POINT('Ctrl Pts',(18.4447331334585,21.756114245197,-9.15227161905073));
#49078=CARTESIAN_POINT('Ctrl Pts',(18.5321062576865,21.7630264334083,-9.15665808106327));
#49079=CARTESIAN_POINT('Ctrl Pts',(18.615438042294,21.7696189066005,-9.1608416525087));
#49080=CARTESIAN_POINT('Ctrl Pts',(18.6992481014932,21.7721377831227,-9.16502522395414));
#49081=CARTESIAN_POINT('Ctrl Pts',(18.7831042309699,21.770529014194,-9.16920879539957));
#49082=CARTESIAN_POINT('Ctrl Pts',(18.8668503855921,21.7689223551186,-9.17338688021374));
#49083=CARTESIAN_POINT('Ctrl Pts',(18.950642035037,21.763198805827,-9.17756496502792));
#49084=CARTESIAN_POINT('Ctrl Pts',(19.0340424954892,21.7533560924663,-9.18174304984209));
#49085=CARTESIAN_POINT('Ctrl Pts',(19.1173586063393,21.7435233338343,-9.18591690902262));
#49086=CARTESIAN_POINT('Ctrl Pts',(19.2002838596484,21.7295797379332,-9.19009076820316));
#49087=CARTESIAN_POINT('Ctrl Pts',(19.2823835816277,21.7115750233499,-9.19426462738369));
#49088=CARTESIAN_POINT('Ctrl Pts',(19.3644249023172,21.6935831163441,-9.19843551750716));
#49089=CARTESIAN_POINT('Ctrl Pts',(19.4456414103873,21.6715359284697,-9.20260640763063));
#49090=CARTESIAN_POINT('Ctrl Pts',(19.5256069084361,21.6455345556217,-9.2067772977541));
#49091=CARTESIAN_POINT('Ctrl Pts',(19.6055553058999,21.6195387431554,-9.21094729593464));
#49092=CARTESIAN_POINT('Ctrl Pts',(19.6842527850321,21.5895905593686,-9.21511729411517));
#49093=CARTESIAN_POINT('Ctrl Pts',(19.7612877178885,21.5558411342083,-9.21928729229571));
#49094=CARTESIAN_POINT('Ctrl Pts',(19.8383126150256,21.5220961057515,-9.22345674723009));
#49095=CARTESIAN_POINT('Ctrl Pts',(19.9136749774785,21.4845510104536,-9.22762620216447));
#49096=CARTESIAN_POINT('Ctrl Pts',(19.9869841268054,21.4434047074788,-9.23179565709885));
#49097=CARTESIAN_POINT('Ctrl Pts',(20.0603319682225,21.4022366877541,-9.23596731264431));
#49098=CARTESIAN_POINT('Ctrl Pts',(20.1316240343934,21.3574638959363,-9.24013896818976));
#49099=CARTESIAN_POINT('Ctrl Pts',(20.2004959726192,21.3093301842874,-9.24431062373522));
#49100=CARTESIAN_POINT('Ctrl Pts',(20.2320270447196,21.287293523616,-9.24622049842687));
#49101=CARTESIAN_POINT('Ctrl Pts',(20.2630512644551,21.2645530061891,-9.24813037311851));
#49102=CARTESIAN_POINT('Ctrl Pts',(20.2935358855687,21.2411349269503,-9.25004024781016));
#49103=CARTESIAN_POINT('Ctrl Pts',(20.2935358855687,21.2411349269503,-8.4501343042798));
#49104=CARTESIAN_POINT('Ctrl Pts',(20.3602160797285,21.1899116539213,-8.45430378913366));
#49105=CARTESIAN_POINT('Ctrl Pts',(20.4243834024368,21.1353894300217,-8.45847327398753));
#49106=CARTESIAN_POINT('Ctrl Pts',(20.4857033606994,21.0778517177629,-8.46264275884139));
#49107=CARTESIAN_POINT('Ctrl Pts',(20.5470302049274,21.0203075442685,-8.46681271191031));
#49108=CARTESIAN_POINT('Ctrl Pts',(20.6055087152443,20.9597475257638,-8.47098266497924));
#49109=CARTESIAN_POINT('Ctrl Pts',(20.6608405095296,20.8964927026943,-8.47515261804817));
#49110=CARTESIAN_POINT('Ctrl Pts',(20.7162314101251,20.8331703098081,-8.47932702552786));
#49111=CARTESIAN_POINT('Ctrl Pts',(20.7684685805212,20.7671477122994,-8.48350143300755));
#49112=CARTESIAN_POINT('Ctrl Pts',(20.8172936334879,20.6987794314578,-8.48767584048725));
#49113=CARTESIAN_POINT('Ctrl Pts',(20.8661466856643,20.630371944149,-8.49185264182222));
#49114=CARTESIAN_POINT('Ctrl Pts',(20.9115834762052,20.5596164825491,-8.49602944315718));
#49115=CARTESIAN_POINT('Ctrl Pts',(20.9533900358615,20.4868949285575,-8.50020624449215));
#49116=CARTESIAN_POINT('Ctrl Pts',(20.9952677481271,20.4140496062299,-8.50439015452768));
#49117=CARTESIAN_POINT('Ctrl Pts',(21.0335026827121,20.3392319193496,-8.50857406456321));
#49118=CARTESIAN_POINT('Ctrl Pts',(21.0679278688898,20.2628463304207,-8.51275797459873));
#49119=CARTESIAN_POINT('Ctrl Pts',(21.0899269822391,20.2140327896478,-8.51543166561785));
#49120=CARTESIAN_POINT('Ctrl Pts',(21.1103712764704,20.1645793566965,-8.51810535663697));
#49121=CARTESIAN_POINT('Ctrl Pts',(21.1292278697972,20.1145947386671,-8.52077904765609));
#49122=CARTESIAN_POINT('Ctrl Pts',(21.1587406102023,20.0363630543649,-8.52496368204914));
#49123=CARTESIAN_POINT('Ctrl Pts',(21.1844714983966,19.9565383690801,-8.52914831644219));
#49124=CARTESIAN_POINT('Ctrl Pts',(21.2062483053234,19.8755211184195,-8.53333295083523));
#49125=CARTESIAN_POINT('Ctrl Pts',(21.227994115661,19.7946191857873,-8.53751162891918));
#49126=CARTESIAN_POINT('Ctrl Pts',(21.2457969056055,19.7125284999513,-8.54169030700313));
#49127=CARTESIAN_POINT('Ctrl Pts',(21.2595330219156,19.6296680728378,-8.54586898508708));
#49128=CARTESIAN_POINT('Ctrl Pts',(21.2735153482386,19.5453224321191,-8.55012256297251));
#49129=CARTESIAN_POINT('Ctrl Pts',(21.2832836065124,19.4601796345795,-8.55437614085795));
#49130=CARTESIAN_POINT('Ctrl Pts',(21.288760950006,19.3746963295992,-8.55862971874338));
#49131=CARTESIAN_POINT('Ctrl Pts',(21.2941321045079,19.290870285293,-8.56280083272133));
#49132=CARTESIAN_POINT('Ctrl Pts',(21.2953772042646,19.206717298763,-8.56697194669928));
#49133=CARTESIAN_POINT('Ctrl Pts',(21.2924758541409,19.1226750104567,-8.57114306067723));
#49134=CARTESIAN_POINT('Ctrl Pts',(21.2895754775933,19.0386609233517,-8.57531277499761));
#49135=CARTESIAN_POINT('Ctrl Pts',(21.2825314303294,18.9547579200745,-8.57948248931798));
#49136=CARTESIAN_POINT('Ctrl Pts',(21.2713754270314,18.8714032651847,-8.58365220363836));
#49137=CARTESIAN_POINT('Ctrl Pts',(21.2602198207119,18.7880515764114,-8.5878217695824));
#49138=CARTESIAN_POINT('Ctrl Pts',(21.2449526111524,18.7052486530836,-8.59199133552644));
#49139=CARTESIAN_POINT('Ctrl Pts',(21.2256571796748,18.6234248992895,-8.59616090147048));
#49140=CARTESIAN_POINT('Ctrl Pts',(21.2056833446299,18.5387243232523,-8.6004770642094));
#49141=CARTESIAN_POINT('Ctrl Pts',(21.181392873751,18.4550735664103,-8.60479322694832));
#49142=CARTESIAN_POINT('Ctrl Pts',(21.1529349892686,18.3729346578625,-8.60910938968724));
#49143=CARTESIAN_POINT('Ctrl Pts',(21.12540411738,18.2934714156211,-8.61328495387892));
#49144=CARTESIAN_POINT('Ctrl Pts',(21.0939733891636,18.2154234566592,-8.61746051807061));
#49145=CARTESIAN_POINT('Ctrl Pts',(21.0588268816571,18.1391884632433,-8.62163608226229));
#49146=CARTESIAN_POINT('Ctrl Pts',(21.0219052076092,18.0591030215416,-8.62602254427483));
#49147=CARTESIAN_POINT('Ctrl Pts',(20.9808827929501,17.981019021216,-8.63040900628737));
#49148=CARTESIAN_POINT('Ctrl Pts',(20.936026279751,17.905365953536,-8.63479546829991));
#49149=CARTESIAN_POINT('Ctrl Pts',(20.8911697665519,17.829712885856,-8.63918193031245));
#49150=CARTESIAN_POINT('Ctrl Pts',(20.842479539431,17.7564911918506,-8.64356839232499));
#49151=CARTESIAN_POINT('Ctrl Pts',(20.790271595083,17.6860911085397,-8.64795485433753));
#49152=CARTESIAN_POINT('Ctrl Pts',(20.7404658156452,17.6189302374198,-8.65213948873058));
#49153=CARTESIAN_POINT('Ctrl Pts',(20.6872735296056,17.5540870442999,-8.65632412312363));
#49154=CARTESIAN_POINT('Ctrl Pts',(20.6309382156176,17.49192309476,-8.66050875751668));
#49155=CARTESIAN_POINT('Ctrl Pts',(20.574683087976,17.4298476279077,-8.66468743560064));
#49156=CARTESIAN_POINT('Ctrl Pts',(20.515294124861,17.370444167647,-8.66886611368458));
#49157=CARTESIAN_POINT('Ctrl Pts',(20.4530567178379,17.3140434899934,-8.67304479176854));
#49158=CARTESIAN_POINT('Ctrl Pts',(20.3897037500234,17.2566318707275,-8.67729836965397));
#49159=CARTESIAN_POINT('Ctrl Pts',(20.3233995043663,17.2023321299324,-8.68155194753941));
#49160=CARTESIAN_POINT('Ctrl Pts',(20.2544863550513,17.1514560591959,-8.68580552542484));
#49161=CARTESIAN_POINT('Ctrl Pts',(20.1869092216086,17.1015663203671,-8.68997663940279));
#49162=CARTESIAN_POINT('Ctrl Pts',(20.1168238263188,17.054968972992,-8.69414775338075));
#49163=CARTESIAN_POINT('Ctrl Pts',(20.0445871160401,17.0119180526252,-8.6983188673587));
#49164=CARTESIAN_POINT('Ctrl Pts',(19.9723746454872,16.9688815784106,-8.70248858167907));
#49165=CARTESIAN_POINT('Ctrl Pts',(19.8980126884862,16.9293894030873,-8.70665829599945));
#49166=CARTESIAN_POINT('Ctrl Pts',(19.8218860818892,16.8936515426394,-8.71082801031982));
#49167=CARTESIAN_POINT('Ctrl Pts',(19.7457621842035,16.8579149538979,-8.71499757626386));
#49168=CARTESIAN_POINT('Ctrl Pts',(19.6678741785624,16.8259326091334,-8.71916714220791));
#49169=CARTESIAN_POINT('Ctrl Pts',(19.5886290994192,16.7978673674193,-8.72333670815195));
#49170=CARTESIAN_POINT('Ctrl Pts',(19.5065978610527,16.7688153864287,-8.72765287089087));
#49171=CARTESIAN_POINT('Ctrl Pts',(19.4231128413864,16.7439612602711,-8.73196903362979));
#49172=CARTESIAN_POINT('Ctrl Pts',(19.338643304938,16.7234296042536,-8.7362851963687));
#49173=CARTESIAN_POINT('Ctrl Pts',(19.2569253547548,16.7035667647714,-8.74046076056038));
#49174=CARTESIAN_POINT('Ctrl Pts',(19.1742865155725,16.6877491532913,-8.74463632475206));
#49175=CARTESIAN_POINT('Ctrl Pts',(19.0911608126521,16.676037248024,-8.74881188894374));
#49176=CARTESIAN_POINT('Ctrl Pts',(19.0038366280897,16.663733802264,-8.75319835095627));
#49177=CARTESIAN_POINT('Ctrl Pts',(18.9159756858735,16.6559617726585,-8.75758481296882));
#49178=CARTESIAN_POINT('Ctrl Pts',(18.8280834484886,16.6527294309005,-8.76197127498135));
#49179=CARTESIAN_POINT('Ctrl Pts',(18.7401912111037,16.6494970891426,-8.76635773699389));
#49180=CARTESIAN_POINT('Ctrl Pts',(18.6522682575722,16.65080435055,-8.77074419900643));
#49181=CARTESIAN_POINT('Ctrl Pts',(18.5648137584889,16.6565967398073,-8.77513066101897));
#49182=CARTESIAN_POINT('Ctrl Pts',(18.481383170547,16.6621226126484,-8.77931529541201));
#49183=CARTESIAN_POINT('Ctrl Pts',(18.3980683312293,16.6717505167586,-8.78349992980506));
#49184=CARTESIAN_POINT('Ctrl Pts',(18.3153050503466,16.6854714337124,-8.78768456419811));
#49185=CARTESIAN_POINT('Ctrl Pts',(18.2326595727499,16.6991728206392,-8.79186324228206));
#49186=CARTESIAN_POINT('Ctrl Pts',(18.1505645441385,16.7169555737484,-8.79604192036602));
#49187=CARTESIAN_POINT('Ctrl Pts',(18.0694525718368,16.7387587666812,-8.80022059844998));
#49188=CARTESIAN_POINT('Ctrl Pts',(17.9868867257259,16.7609527661775,-8.80447417633541));
#49189=CARTESIAN_POINT('Ctrl Pts',(17.9053400062228,16.7873127240844,-8.80872775422085));
#49190=CARTESIAN_POINT('Ctrl Pts',(17.8252599013632,16.8177195247674,-8.81298133210628));
#49191=CARTESIAN_POINT('Ctrl Pts',(17.7467323055997,16.8475368302852,-8.81715244608423));
#49192=CARTESIAN_POINT('Ctrl Pts',(17.6696154154516,16.8812452961241,-8.82132356006219));
#49193=CARTESIAN_POINT('Ctrl Pts',(17.5943160431827,16.918682291092,-8.82549467404014));
#49194=CARTESIAN_POINT('Ctrl Pts',(17.5190419383454,16.9561067237147,-8.82966438836052));
#49195=CARTESIAN_POINT('Ctrl Pts',(17.4455845517321,16.9972569960436,-8.83383410268089));
#49196=CARTESIAN_POINT('Ctrl Pts',(17.3743287784388,17.0419231988567,-8.83800381700126));
#49197=CARTESIAN_POINT('Ctrl Pts',(17.3030755407317,17.0865878122545,-8.8421733829453));
#49198=CARTESIAN_POINT('Ctrl Pts',(17.23402414991,17.1347678623266,-8.84634294888934));
#49199=CARTESIAN_POINT('Ctrl Pts',(17.1675318647109,17.18620925004,-8.85051251483338));
#49200=CARTESIAN_POINT('Ctrl Pts',(17.0987017927912,17.2394592534855,-8.8548286775723));
#49201=CARTESIAN_POINT('Ctrl Pts',(17.0326145482166,17.2962038761407,-8.85914484031122));
#49202=CARTESIAN_POINT('Ctrl Pts',(16.9696289167229,17.3561159927113,-8.86346100305014));
#49203=CARTESIAN_POINT('Ctrl Pts',(16.9086950355501,17.4140764783862,-8.86763656724182));
#49204=CARTESIAN_POINT('Ctrl Pts',(16.8506640912069,17.4750008911692,-8.87181213143349));
#49205=CARTESIAN_POINT('Ctrl Pts',(16.795821865939,17.5385570202103,-8.87598769562517));
#49206=CARTESIAN_POINT('Ctrl Pts',(16.738209690248,17.6053232182388,-8.88037415763771));
#49207=CARTESIAN_POINT('Ctrl Pts',(16.684117181693,17.6749935141298,-8.88476061965025));
#49208=CARTESIAN_POINT('Ctrl Pts',(16.6338248927154,17.747147371235,-8.88914708166279));
#49209=CARTESIAN_POINT('Ctrl Pts',(16.5835326037379,17.8193012283402,-8.89353354367533));
#49210=CARTESIAN_POINT('Ctrl Pts',(16.5370407765469,17.8939381139568,-8.89792000568786));
#49211=CARTESIAN_POINT('Ctrl Pts',(16.4945737975988,17.9706088181549,-8.9023064677004));
#49212=CARTESIAN_POINT('Ctrl Pts',(16.4520961746313,18.0472987392713,-8.90669402914567));
#49213=CARTESIAN_POINT('Ctrl Pts',(16.4134992022808,18.1262856298358,-8.91108159059094));
#49214=CARTESIAN_POINT('Ctrl Pts',(16.3790251742671,18.2071605854698,-8.91546915203621));
#49215=CARTESIAN_POINT('Ctrl Pts',(16.3446454932945,18.2878142059945,-8.91984470579152));
#49216=CARTESIAN_POINT('Ctrl Pts',(16.3143664333072,18.3703452363826,-8.92422025954683));
#49217=CARTESIAN_POINT('Ctrl Pts',(16.2883841141658,18.4543211123896,-8.92859581330214));
#49218=CARTESIAN_POINT('Ctrl Pts',(16.2624439986578,18.5381605845957,-8.93296425975245));
#49219=CARTESIAN_POINT('Ctrl Pts',(16.2407868563187,18.6234398583863,-8.93733270620276));
#49220=CARTESIAN_POINT('Ctrl Pts',(16.2235607960525,18.7097066694205,-8.94170115265307));
#49221=CARTESIAN_POINT('Ctrl Pts',(16.2063704951607,18.7957944002037,-8.94606053069715));
#49222=CARTESIAN_POINT('Ctrl Pts',(16.193593030381,18.8828651985171,-8.95041990874122));
#49223=CARTESIAN_POINT('Ctrl Pts',(16.1853263642748,18.9704533339262,-8.9547792867853));
#49224=CARTESIAN_POINT('Ctrl Pts',(16.1777850503447,19.0503561166421,-8.9587561545997));
#49225=CARTESIAN_POINT('Ctrl Pts',(16.1739971536887,19.1306890276032,-8.96273302241411));
#49226=CARTESIAN_POINT('Ctrl Pts',(16.174000001606,19.21109067809,-8.96670989022851));
#49227=CARTESIAN_POINT('Origin',(18.734,19.211,1.76670989022852));
#49228=CARTESIAN_POINT('',(20.2947700725713,21.2427129721482,-7.6502134855505));
#49229=CARTESIAN_POINT('',(20.2923705327637,21.2395869487749,-7.71658757605019));
#49230=CARTESIAN_POINT('',(20.2935358855687,21.2411349269503,1.76670989022852));
#49231=CARTESIAN_POINT('',(16.1740010826189,19.2133543592346,-8.23329012251325));
#49232=CARTESIAN_POINT('Ctrl Pts',(20.2923705327634,21.239586948775,-7.71658757605017));
#49233=CARTESIAN_POINT('Ctrl Pts',(20.5052428186746,21.0789785260141,-7.72982826792657));
#49234=CARTESIAN_POINT('Ctrl Pts',(21.2942513389235,20.2707707462439,-7.78546089536344));
#49235=CARTESIAN_POINT('Ctrl Pts',(21.5288884363408,18.0482922871128,-7.88348545836079));
#49236=CARTESIAN_POINT('Ctrl Pts',(19.2691669172862,16.2315894932317,-8.01066126504223));
#49237=CARTESIAN_POINT('Ctrl Pts',(16.7471750875427,17.0720885005601,-8.12726281551246));
#49238=CARTESIAN_POINT('Ctrl Pts',(16.180230297531,18.573538664413,-8.20147243042223));
#49239=CARTESIAN_POINT('Ctrl Pts',(16.1744184457826,19.2133537191784,-8.23329010977151));
#49240=CARTESIAN_POINT('Ctrl Pts',(16.1740010826189,19.2133543592346,-8.23329012251325));
#49241=CARTESIAN_POINT('Ctrl Pts',(16.1741014808466,19.322521792358,-8.23871812867197));
#49242=CARTESIAN_POINT('Ctrl Pts',(16.1811885397039,19.4313771444072,-8.24414613483068));
#49243=CARTESIAN_POINT('Ctrl Pts',(16.1951208364047,19.5391654958424,-8.2495741409894));
#49244=CARTESIAN_POINT('Ctrl Pts',(16.2083299266963,19.6413587018203,-8.25472038679463));
#49245=CARTESIAN_POINT('Ctrl Pts',(16.2276915596972,19.7425933354954,-8.25986663259986));
#49246=CARTESIAN_POINT('Ctrl Pts',(16.253046772176,19.84224565848,-8.2650128784051));
#49247=CARTESIAN_POINT('Ctrl Pts',(16.2736641888712,19.9232772597465,-8.26919751279815));
#49248=CARTESIAN_POINT('Ctrl Pts',(16.2982940662942,20.0034485022604,-8.27338214719119));
#49249=CARTESIAN_POINT('Ctrl Pts',(16.3268482220627,20.0823324956487,-8.27756678158424));
#49250=CARTESIAN_POINT('Ctrl Pts',(16.3553617345248,20.1611042074361,-8.28174545966818));
#49251=CARTESIAN_POINT('Ctrl Pts',(16.3877882750863,20.2385918806365,-8.28592413775212));
#49252=CARTESIAN_POINT('Ctrl Pts',(16.4239892031399,20.314381220789,-8.29010281583606));
#49253=CARTESIAN_POINT('Ctrl Pts',(16.4608390068118,20.3915290303949,-8.2943563937215));
#49254=CARTESIAN_POINT('Ctrl Pts',(16.5015997218018,20.4669165555969,-8.29860997160693));
#49255=CARTESIAN_POINT('Ctrl Pts',(16.5460727818105,20.5401254598065,-8.30286354949237));
#49256=CARTESIAN_POINT('Ctrl Pts',(16.589683644769,20.6119150665525,-8.30703466347032));
#49257=CARTESIAN_POINT('Ctrl Pts',(16.6368639453122,20.6816093608382,-8.31120577744827));
#49258=CARTESIAN_POINT('Ctrl Pts',(16.6873797310322,20.7488379221005,-8.31537689142623));
#49259=CARTESIAN_POINT('Ctrl Pts',(16.7378785656925,20.8160439241698,-8.3195466057466));
#49260=CARTESIAN_POINT('Ctrl Pts',(16.7917103865529,20.880785468974,-8.32371632006697));
#49261=CARTESIAN_POINT('Ctrl Pts',(16.8485987415145,20.9427222913912,-8.32788603438734));
#49262=CARTESIAN_POINT('Ctrl Pts',(16.9054850721443,21.0046569098304,-8.33205560033138));
#49263=CARTESIAN_POINT('Ctrl Pts',(16.9654274088046,21.0637866660879,-8.33622516627543));
#49264=CARTESIAN_POINT('Ctrl Pts',(17.0281108772059,21.1198065121255,-8.34039473221947));
#49265=CARTESIAN_POINT('Ctrl Pts',(17.0929982190277,21.1777959468418,-8.34471089495839));
#49266=CARTESIAN_POINT('Ctrl Pts',(17.160822642128,21.2324523620817,-8.34902705769731));
#49267=CARTESIAN_POINT('Ctrl Pts',(17.2311971876102,21.2834824986169,-8.35334322043623));
#49268=CARTESIAN_POINT('Ctrl Pts',(17.2992792896755,21.3328503338219,-8.35751878462791));
#49269=CARTESIAN_POINT('Ctrl Pts',(17.3697475047295,21.3788242964685,-8.36169434881959));
#49270=CARTESIAN_POINT('Ctrl Pts',(17.4422231594135,21.4211838371783,-8.36586991301127));
#49271=CARTESIAN_POINT('Ctrl Pts',(17.5183593871211,21.4656828575892,-8.37025637502381));
#49272=CARTESIAN_POINT('Ctrl Pts',(17.5967106568092,21.5061924632349,-8.37464283703636));
#49273=CARTESIAN_POINT('Ctrl Pts',(17.6768123961765,21.5425133219267,-8.3790292990489));
#49274=CARTESIAN_POINT('Ctrl Pts',(17.7569141355438,21.5788341806186,-8.38341576106144));
#49275=CARTESIAN_POINT('Ctrl Pts',(17.8387657767031,21.6109661511407,-8.38780222307398));
#49276=CARTESIAN_POINT('Ctrl Pts',(17.921884774769,21.638770347654,-8.39218868508652));
#49277=CARTESIAN_POINT('Ctrl Pts',(18.0011804710188,21.6652956086952,-8.3963733789285));
#49278=CARTESIAN_POINT('Ctrl Pts',(18.0819246518068,21.6879812201688,-8.40055807277047));
#49279=CARTESIAN_POINT('Ctrl Pts',(18.1637106209527,21.7066702554917,-8.40474276661245));
#49280=CARTESIAN_POINT('Ctrl Pts',(18.2453798597931,21.7253326165961,-8.40892148778459));
#49281=CARTESIAN_POINT('Ctrl Pts',(18.3280874888049,21.7400096304256,-8.41310020895674));
#49282=CARTESIAN_POINT('Ctrl Pts',(18.4114100949888,21.7505936196929,-8.41727893012888));
#49283=CARTESIAN_POINT('Ctrl Pts',(18.4946347461077,21.7611651662942,-8.4214527387458));
#49284=CARTESIAN_POINT('Ctrl Pts',(18.5784724833061,21.7676531957144,-8.42562654736272));
#49285=CARTESIAN_POINT('Ctrl Pts',(18.6624895012298,21.7700010255109,-8.42980035597964));
#49286=CARTESIAN_POINT('Ctrl Pts',(18.7464521744715,21.7723473366619,-8.4339714648542));
#49287=CARTESIAN_POINT('Ctrl Pts',(18.8305934396791,21.7705587522909,-8.43814257372877));
#49288=CARTESIAN_POINT('Ctrl Pts',(18.9144752300251,21.764630492328,-8.44231368260333));
#49289=CARTESIAN_POINT('Ctrl Pts',(18.9983279261209,21.7587042885716,-8.44648334473617));
#49290=CARTESIAN_POINT('Ctrl Pts',(19.0819208676515,21.7486412935491,-8.45065300686901));
#49291=CARTESIAN_POINT('Ctrl Pts',(19.1648182224781,21.7344887872112,-8.45482266900186));
#49292=CARTESIAN_POINT('Ctrl Pts',(19.2477116915592,21.7203369442605,-8.4589921356852));
#49293=CARTESIAN_POINT('Ctrl Pts',(19.3299091855241,21.7020960496226,-8.46316160236854));
#49294=CARTESIAN_POINT('Ctrl Pts',(19.4109835709537,21.6798647684024,-8.46733106905189));
#49295=CARTESIAN_POINT('Ctrl Pts',(19.4921313337435,21.6576133664903,-8.47150430936184));
#49296=CARTESIAN_POINT('Ctrl Pts',(19.5721535125693,21.6313644844617,-8.4756775496718));
#49297=CARTESIAN_POINT('Ctrl Pts',(19.6506371967119,21.601266982913,-8.47985078998176));
#49298=CARTESIAN_POINT('Ctrl Pts',(19.7291549023672,21.5711564345439,-8.48402583932947));
#49299=CARTESIAN_POINT('Ctrl Pts',(19.8061323627767,21.537194127788,-8.48820088867719));
#49300=CARTESIAN_POINT('Ctrl Pts',(19.8811779671275,21.4995765689042,-8.4923759380249));
#49301=CARTESIAN_POINT('Ctrl Pts',(19.9563509512632,21.4618951592911,-8.49655807395541));
#49302=CARTESIAN_POINT('Ctrl Pts',(20.0295851250182,21.4205463259095,-8.50074020988591));
#49303=CARTESIAN_POINT('Ctrl Pts',(20.1005148649941,21.3757718410378,-8.50492234581642));
#49304=CARTESIAN_POINT('Ctrl Pts',(20.1669693717355,21.3338223526038,-8.50884061452122));
#49305=CARTESIAN_POINT('Ctrl Pts',(20.2314010883057,21.2888664569032,-8.51275888322602));
#49306=CARTESIAN_POINT('Ctrl Pts',(20.2935358855687,21.2411349269503,-8.51667715193082));
#49307=CARTESIAN_POINT('',(16.1740010575059,19.2086731074563,-8.16670989022852));
#49308=CARTESIAN_POINT('Ctrl Pts',(16.1740010575059,19.2086731074563,-8.16670989022852));
#49309=CARTESIAN_POINT('Ctrl Pts',(16.1739251952239,19.2921352174732,-8.17086478789788));
#49310=CARTESIAN_POINT('Ctrl Pts',(16.1779353066412,19.375721983002,-8.17501968556725));
#49311=CARTESIAN_POINT('Ctrl Pts',(16.1860403077383,19.458994771335,-8.17917458323661));
#49312=CARTESIAN_POINT('Ctrl Pts',(16.1940671586084,19.5414646248839,-8.18328941845664));
#49313=CARTESIAN_POINT('Ctrl Pts',(16.206110236511,19.6236260477268,-8.18740425367667));
#49314=CARTESIAN_POINT('Ctrl Pts',(16.2221259449782,19.7050533692914,-8.1915190888967));
#49315=CARTESIAN_POINT('Ctrl Pts',(16.238134689091,19.7864452825742,-8.19563213480029));
#49316=CARTESIAN_POINT('Ctrl Pts',(16.2581125446655,19.8671032636359,-8.19974518070388));
#49317=CARTESIAN_POINT('Ctrl Pts',(16.2819644394347,19.9466096857188,-8.20385822660747));
#49318=CARTESIAN_POINT('Ctrl Pts',(16.3058135810413,20.0261069305807,-8.20797079775279));
#49319=CARTESIAN_POINT('Ctrl Pts',(16.3335357367831,20.1044524267965,-8.21208336889812));
#49320=CARTESIAN_POINT('Ctrl Pts',(16.364985800536,20.1812431255815,-8.21619594004344));
#49321=CARTESIAN_POINT('Ctrl Pts',(16.3969970744394,20.2594041147404,-8.22038189789759));
#49322=CARTESIAN_POINT('Ctrl Pts',(16.4328704281986,20.3359537977656,-8.22456785575174));
#49323=CARTESIAN_POINT('Ctrl Pts',(16.4724022025115,20.4104896424709,-8.22875381360589));
#49324=CARTESIAN_POINT('Ctrl Pts',(16.5112918107484,20.4838147044136,-8.23287177349698));
#49325=CARTESIAN_POINT('Ctrl Pts',(16.5537215594669,20.555190490736,-8.23698973338807));
#49326=CARTESIAN_POINT('Ctrl Pts',(16.5994527799559,20.6242615346786,-8.24110769327916));
#49327=CARTESIAN_POINT('Ctrl Pts',(16.6463167081171,20.6950433858238,-8.24532765011484));
#49328=CARTESIAN_POINT('Ctrl Pts',(16.696647513794,20.7634043768934,-8.24954760695052));
#49329=CARTESIAN_POINT('Ctrl Pts',(16.7501447185242,20.828998214511,-8.2537675637862));
#49330=CARTESIAN_POINT('Ctrl Pts',(16.8036419232544,20.8945920521286,-8.25798752062187));
#49331=CARTESIAN_POINT('Ctrl Pts',(16.8603051182411,20.9574183953713,-8.26220747745755));
#49332=CARTESIAN_POINT('Ctrl Pts',(16.9197953580223,21.0171731691692,-8.26642743429323));
#49333=CARTESIAN_POINT('Ctrl Pts',(16.9787876447051,21.0764277756308,-8.27061206868628));
#49334=CARTESIAN_POINT('Ctrl Pts',(17.0407957809271,21.1328994502154,-8.27479670307933));
#49335=CARTESIAN_POINT('Ctrl Pts',(17.1055265727616,21.1862656268913,-8.27898133747238));
#49336=CARTESIAN_POINT('Ctrl Pts',(17.1701652283259,21.2395558434201,-8.28316001555632));
#49337=CARTESIAN_POINT('Ctrl Pts',(17.237518489892,21.2897490519968,-8.28733869364026));
#49338=CARTESIAN_POINT('Ctrl Pts',(17.3072561423604,21.3365592122281,-8.29151737172421));
#49339=CARTESIAN_POINT('Ctrl Pts',(17.3782437921299,21.3842084109397,-8.29577094960964));
#49340=CARTESIAN_POINT('Ctrl Pts',(17.4517018138302,21.4283517444167,-8.30002452749508));
#49341=CARTESIAN_POINT('Ctrl Pts',(17.5272463530812,21.4687301954946,-8.30427810538051));
#49342=CARTESIAN_POINT('Ctrl Pts',(17.6013263140258,21.5083258315063,-8.30844921935846));
#49343=CARTESIAN_POINT('Ctrl Pts',(17.6774121876524,21.5443010347691,-8.31262033333642));
#49344=CARTESIAN_POINT('Ctrl Pts',(17.75511405008,21.5764560442014,-8.31679144731437));
#49345=CARTESIAN_POINT('Ctrl Pts',(17.8327898388973,21.6086002637098,-8.32096116163474));
#49346=CARTESIAN_POINT('Ctrl Pts',(17.9120801148579,21.6369266595075,-8.32513087595512));
#49347=CARTESIAN_POINT('Ctrl Pts',(17.9925737212262,21.6612830598002,-8.32930059027549));
#49348=CARTESIAN_POINT('Ctrl Pts',(18.0730644632864,21.6856385933875,-8.33347015621953));
#49349=CARTESIAN_POINT('Ctrl Pts',(18.1547580100543,21.7060242799309,-8.33763972216357));
#49350=CARTESIAN_POINT('Ctrl Pts',(18.2372280581078,21.7223378183249,-8.34180928810762));
#49351=CARTESIAN_POINT('Ctrl Pts',(18.3225976513131,21.7392249206038,-8.34612545084654));
#49352=CARTESIAN_POINT('Ctrl Pts',(18.4087988479273,21.7517480910506,-8.35044161358546));
#49353=CARTESIAN_POINT('Ctrl Pts',(18.4953492973482,21.7598518674344,-8.35475777632438));
#49354=CARTESIAN_POINT('Ctrl Pts',(18.5790803749826,21.7676916641549,-8.35893334051605));
#49355=CARTESIAN_POINT('Ctrl Pts',(18.6631378283657,21.7713955951849,-8.36310890470773));
#49356=CARTESIAN_POINT('Ctrl Pts',(18.7470834485355,21.770966566847,-8.36728446889941));
#49357=CARTESIAN_POINT('Ctrl Pts',(18.8352689624184,21.7705158693077,-8.37167093091195));
#49358=CARTESIAN_POINT('Ctrl Pts',(18.9233304658568,21.7655037616187,-8.3760573929245));
#49359=CARTESIAN_POINT('Ctrl Pts',(19.0107666109435,21.7559951361578,-8.38044385493704));
#49360=CARTESIAN_POINT('Ctrl Pts',(19.0982027560302,21.7464865106969,-8.38483031694958));
#49361=CARTESIAN_POINT('Ctrl Pts',(19.1850129820694,21.7324815349687,-8.38921677896212));
#49362=CARTESIAN_POINT('Ctrl Pts',(19.2707112385803,21.7141062794819,-8.39360324097466));
#49363=CARTESIAN_POINT('Ctrl Pts',(19.3524727077245,21.6965751423775,-8.39778819867499));
#49364=CARTESIAN_POINT('Ctrl Pts',(19.4335264843041,21.67500117954,-8.40197315637533));
#49365=CARTESIAN_POINT('Ctrl Pts',(19.5134425416024,21.6494563404622,-8.40615811407565));
#49366=CARTESIAN_POINT('Ctrl Pts',(19.5932250321231,21.6239541954556,-8.41033607729536));
#49367=CARTESIAN_POINT('Ctrl Pts',(19.6718731494994,21.5944945081295,-8.41451404051505));
#49368=CARTESIAN_POINT('Ctrl Pts',(19.7489678548335,21.5612000454546,-8.41869200373476));
#49369=CARTESIAN_POINT('Ctrl Pts',(19.8259879712299,21.5279377950904,-8.42286592478533));
#49370=CARTESIAN_POINT('Ctrl Pts',(19.9014572393319,21.4908483161393,-8.4270398458359));
#49371=CARTESIAN_POINT('Ctrl Pts',(19.9749733693948,21.4501036368272,-8.43121376688647));
#49372=CARTESIAN_POINT('Ctrl Pts',(20.048437496638,21.4093877789209,-8.43538473544669));
#49373=CARTESIAN_POINT('Ctrl Pts',(20.1199508294576,21.3650220797911,-8.43955570400692));
#49374=CARTESIAN_POINT('Ctrl Pts',(20.1891338986603,21.3172253765848,-8.44372667256715));
#49375=CARTESIAN_POINT('Ctrl Pts',(20.2245612917467,21.2927495530598,-8.4458625498047));
#49376=CARTESIAN_POINT('Ctrl Pts',(20.2593780186155,21.2673747687365,-8.44799842704225));
#49377=CARTESIAN_POINT('Ctrl Pts',(20.2935358855687,21.2411349269503,-8.4501343042798));
#49378=CARTESIAN_POINT('Ctrl Pts',(20.2947700725713,21.2427129721481,-7.65021348555051));
#49379=CARTESIAN_POINT('Ctrl Pts',(20.8607342680588,20.7994053635694,-7.6860503928895));
#49380=CARTESIAN_POINT('Ctrl Pts',(21.6914150496944,19.288541779014,-7.76427923578897));
#49381=CARTESIAN_POINT('Ctrl Pts',(20.5479111384388,16.787568886273,-7.88490001424893));
#49382=CARTESIAN_POINT('Ctrl Pts',(17.6781136453352,16.37403049238,-8.01207582093036));
#49383=CARTESIAN_POINT('Ctrl Pts',(16.2739021846612,17.9910560858828,-8.10601244625689));
#49384=CARTESIAN_POINT('Ctrl Pts',(16.1718447049445,19.0247813383249,-8.15755713602294));
#49385=CARTESIAN_POINT('Ctrl Pts',(16.1735502234357,19.2086726976739,-8.16670989022852));
#49386=CARTESIAN_POINT('Origin',(18.734,19.211,1.76670989022852));
#49387=CARTESIAN_POINT('',(20.2935358855687,21.2411349269503,-6.85004462256371));
#49388=CARTESIAN_POINT('',(20.2935358855687,21.2411349269503,-6.91673142315837));
#49389=CARTESIAN_POINT('',(20.2935358855687,21.2411349269503,1.76670989022852));
#49390=CARTESIAN_POINT('',(16.1743644999821,19.2104398261047,-7.43329008494582));
#49391=CARTESIAN_POINT('Ctrl Pts',(20.2935358855687,21.2411349269503,-6.91673142315837));
#49392=CARTESIAN_POINT('Ctrl Pts',(20.3602014276152,21.1899229095753,-6.92090111997205));
#49393=CARTESIAN_POINT('Ctrl Pts',(20.4243665511424,21.1354046687238,-6.92507081678572));
#49394=CARTESIAN_POINT('Ctrl Pts',(20.4856940824214,21.0778604237087,-6.9292405135994));
#49395=CARTESIAN_POINT('Ctrl Pts',(20.5470198554989,21.0203178284319,-6.93341009087187));
#49396=CARTESIAN_POINT('Ctrl Pts',(20.6055078632375,20.9597497169416,-6.93757966814435));
#49397=CARTESIAN_POINT('Ctrl Pts',(20.6608565789692,20.8964743320748,-6.94174924541683));
#49398=CARTESIAN_POINT('Ctrl Pts',(20.7178321177842,20.8313391415135,-6.94604137593132));
#49399=CARTESIAN_POINT('Ctrl Pts',(20.7714805809141,20.7633354172175,-6.95033350644581));
#49400=CARTESIAN_POINT('Ctrl Pts',(20.8215177086802,20.6928467585909,-6.95462563696031));
#49401=CARTESIAN_POINT('Ctrl Pts',(20.8701964139745,20.6242717465336,-6.95880124346946));
#49402=CARTESIAN_POINT('Ctrl Pts',(20.9154571725214,20.5533454368994,-6.96297684997862));
#49403=CARTESIAN_POINT('Ctrl Pts',(20.9570834048037,20.4804487682795,-6.96715245648777));
#49404=CARTESIAN_POINT('Ctrl Pts',(21.0004520625165,20.404500730313,-6.97150284900493));
#49405=CARTESIAN_POINT('Ctrl Pts',(21.0398749854783,20.3264142577069,-6.9758532415221));
#49406=CARTESIAN_POINT('Ctrl Pts',(21.0751622346957,20.2466444326285,-6.98020363403926));
#49407=CARTESIAN_POINT('Ctrl Pts',(21.1104494839132,20.1668746075502,-6.98455402655642));
#49408=CARTESIAN_POINT('Ctrl Pts',(21.1416009291318,20.0854219761771,-6.98890441907358));
#49409=CARTESIAN_POINT('Ctrl Pts',(21.1684852750765,20.0027584514458,-6.99325481159075));
#49410=CARTESIAN_POINT('Ctrl Pts',(21.1943452769569,19.9232445622331,-6.99743944598379));
#49411=CARTESIAN_POINT('Ctrl Pts',(21.2163537449119,19.8423144298574,-7.00162408037684));
#49412=CARTESIAN_POINT('Ctrl Pts',(21.234357169427,19.7603760326907,-7.00580871476988));
#49413=CARTESIAN_POINT('Ctrl Pts',(21.2523349682956,19.6785542646905,-7.00998739285382));
#49414=CARTESIAN_POINT('Ctrl Pts',(21.2663189491972,19.5957275280113,-7.01416607093776));
#49415=CARTESIAN_POINT('Ctrl Pts',(21.2762049862094,19.5123201090075,-7.0183447490217));
#49416=CARTESIAN_POINT('Ctrl Pts',(21.28626822333,19.4274176719618,-7.02259832690713));
#49417=CARTESIAN_POINT('Ctrl Pts',(21.2920850111441,19.3419139888709,-7.02685190479257));
#49418=CARTESIAN_POINT('Ctrl Pts',(21.2935997221946,19.2562687766723,-7.031105482678));
#49419=CARTESIAN_POINT('Ctrl Pts',(21.2950850676157,19.1722839640351,-7.03527659665596));
#49420=CARTESIAN_POINT('Ctrl Pts',(21.2924336475013,19.088163542099,-7.03944771063391));
#49421=CARTESIAN_POINT('Ctrl Pts',(21.2856453456189,19.0043456262704,-7.04361882461186));
#49422=CARTESIAN_POINT('Ctrl Pts',(21.2788593216167,18.9205558363528,-7.04778853893223));
#49423=CARTESIAN_POINT('Ctrl Pts',(21.2679392098804,18.8370688090943,-7.05195825325261));
#49424=CARTESIAN_POINT('Ctrl Pts',(21.252936930744,18.7543198724117,-7.05612796757298));
#49425=CARTESIAN_POINT('Ctrl Pts',(21.2379351854531,18.6715738802915,-7.06029753351703));
#49426=CARTESIAN_POINT('Ctrl Pts',(21.2188516444825,18.5895663790285,-7.06446709946107));
#49427=CARTESIAN_POINT('Ctrl Pts',(21.1957895218785,18.5087234519298,-7.06863666540511));
#49428=CARTESIAN_POINT('Ctrl Pts',(21.1719165634939,18.4250381872448,-7.07295282814404));
#49429=CARTESIAN_POINT('Ctrl Pts',(21.1437801888442,18.3426014204637,-7.07726899088296));
#49430=CARTESIAN_POINT('Ctrl Pts',(21.1115508461405,18.261867778433,-7.08158515362188));
#49431=CARTESIAN_POINT('Ctrl Pts',(21.0803713708855,18.1837640263,-7.08576071781356));
#49432=CARTESIAN_POINT('Ctrl Pts',(21.0453617283798,18.1072545529914,-7.08993628200524));
#49433=CARTESIAN_POINT('Ctrl Pts',(21.006724205865,18.032728094167,-7.09411184619691));
#49434=CARTESIAN_POINT('Ctrl Pts',(20.9661351939398,17.9544374810769,-7.09849830820946));
#49435=CARTESIAN_POINT('Ctrl Pts',(20.9215424772638,17.8783359749763,-7.102884770222));
#49436=CARTESIAN_POINT('Ctrl Pts',(20.8732322919594,17.8048402647501,-7.10727123223455));
#49437=CARTESIAN_POINT('Ctrl Pts',(20.8249221066551,17.731344554524,-7.11165769424709));
#49438=CARTESIAN_POINT('Ctrl Pts',(20.7728948573422,17.6604550629257,-7.11604415625964));
#49439=CARTESIAN_POINT('Ctrl Pts',(20.7174842649081,17.5925469821889,-7.12043061827219));
#49440=CARTESIAN_POINT('Ctrl Pts',(20.6646231959702,17.5277634529108,-7.12461525266524));
#49441=CARTESIAN_POINT('Ctrl Pts',(20.6084865283937,17.4654518685825,-7.12879988705828));
#49442=CARTESIAN_POINT('Ctrl Pts',(20.549334215637,17.4059621373673,-7.13298452145133));
#49443=CARTESIAN_POINT('Ctrl Pts',(20.4902660988757,17.3465570824209,-7.13716319953529));
#49444=CARTESIAN_POINT('Ctrl Pts',(20.4281911845783,17.2899662258643,-7.14134187761925));
#49445=CARTESIAN_POINT('Ctrl Pts',(20.3634098690371,17.2365067792762,-7.1455205557032));
#49446=CARTESIAN_POINT('Ctrl Pts',(20.2974673949727,17.1820891105288,-7.14977413358864));
#49447=CARTESIAN_POINT('Ctrl Pts',(20.2287208456641,17.1309165905524,-7.15402771147407));
#49448=CARTESIAN_POINT('Ctrl Pts',(20.1575266602167,17.083284829294,-7.15828128935951));
#49449=CARTESIAN_POINT('Ctrl Pts',(20.0877127129782,17.0365765026734,-7.16245240333746));
#49450=CARTESIAN_POINT('Ctrl Pts',(20.0155455870556,16.9932731384694,-7.1666235173154));
#49451=CARTESIAN_POINT('Ctrl Pts',(19.9413936052579,16.9536119779749,-7.17079463129335));
#49452=CARTESIAN_POINT('Ctrl Pts',(19.8672665058736,16.9139641261658,-7.17496434561373));
#49453=CARTESIAN_POINT('Ctrl Pts',(19.7911562786912,16.8779562675926,-7.1791340599341));
#49454=CARTESIAN_POINT('Ctrl Pts',(19.7134570690884,16.8457803802157,-7.18330377425448));
#49455=CARTESIAN_POINT('Ctrl Pts',(19.6357606243572,16.8136056377949,-7.18747334019852));
#49456=CARTESIAN_POINT('Ctrl Pts',(19.5564757349841,16.7852627706771,-7.19164290614255));
#49457=CARTESIAN_POINT('Ctrl Pts',(19.476016537407,16.7608956229959,-7.19581247208659));
#49458=CARTESIAN_POINT('Ctrl Pts',(19.3927284937001,16.7356717564624,-7.20012863482551));
#49459=CARTESIAN_POINT('Ctrl Pts',(19.3081825327891,16.7147085365433,-7.20444479756443));
#49460=CARTESIAN_POINT('Ctrl Pts',(19.2228531842896,16.6981087241566,-7.20876096030335));
#49461=CARTESIAN_POINT('Ctrl Pts',(19.1403034303422,16.6820496489123,-7.21293652449504));
#49462=CARTESIAN_POINT('Ctrl Pts',(19.0570210156983,16.6700740910786,-7.21711208868672));
#49463=CARTESIAN_POINT('Ctrl Pts',(18.9734422997759,16.6622223743374,-7.2212876528784));
#49464=CARTESIAN_POINT('Ctrl Pts',(18.8856422216019,16.6539740860494,-7.22567411489094));
#49465=CARTESIAN_POINT('Ctrl Pts',(18.7975157065269,16.6502772019506,-7.23006057690348));
#49466=CARTESIAN_POINT('Ctrl Pts',(18.7095680581451,16.6511165885499,-7.23444703891601));
#49467=CARTESIAN_POINT('Ctrl Pts',(18.6216204097632,16.6519559751493,-7.23883350092855));
#49468=CARTESIAN_POINT('Ctrl Pts',(18.5338522025563,16.6573315210541,-7.24321996294108));
#49469=CARTESIAN_POINT('Ctrl Pts',(18.4467595506041,16.6671657042506,-7.24760642495362));
#49470=CARTESIAN_POINT('Ctrl Pts',(18.3636741606704,16.6765474021004,-7.25179105934667));
#49471=CARTESIAN_POINT('Ctrl Pts',(18.2808942658293,16.6900213769478,-7.25597569373972));
#49472=CARTESIAN_POINT('Ctrl Pts',(18.1988547913486,16.7075584477249,-7.26016032813276));
#49473=CARTESIAN_POINT('Ctrl Pts',(18.116932089905,16.7250705566525,-7.26433900621672));
#49474=CARTESIAN_POINT('Ctrl Pts',(18.0357481614728,16.7466341786849,-7.26851768430067));
#49475=CARTESIAN_POINT('Ctrl Pts',(17.9557323296054,16.77216842869,-7.27269636238463));
#49476=CARTESIAN_POINT('Ctrl Pts',(17.8742822714585,16.7981603617751,-7.27694994027006));
#49477=CARTESIAN_POINT('Ctrl Pts',(17.7940430771259,16.8282666158667,-7.2812035181555));
#49478=CARTESIAN_POINT('Ctrl Pts',(17.7154562415191,16.8623474901426,-7.28545709604093));
#49479=CARTESIAN_POINT('Ctrl Pts',(17.63839296507,16.8957676401673,-7.28962821001889));
#49480=CARTESIAN_POINT('Ctrl Pts',(17.5629189921761,16.9330094826425,-7.29379932399685));
#49481=CARTESIAN_POINT('Ctrl Pts',(17.4894331713713,16.9738917305867,-7.2979704379748));
#49482=CARTESIAN_POINT('Ctrl Pts',(17.4159720094435,17.0147602600978,-7.30214015229517));
#49483=CARTESIAN_POINT('Ctrl Pts',(17.3444980763215,17.059266545551,-7.30630986661554));
#49484=CARTESIAN_POINT('Ctrl Pts',(17.2753861385062,17.1071830870871,-7.31047958093591));
#49485=CARTESIAN_POINT('Ctrl Pts',(17.2062766599905,17.155097923547,-7.31464914687994));
#49486=CARTESIAN_POINT('Ctrl Pts',(17.1395293872397,17.2064225119979,-7.31881871282397));
#49487=CARTESIAN_POINT('Ctrl Pts',(17.0754894346056,17.2608864893358,-7.322988278768));
#49488=CARTESIAN_POINT('Ctrl Pts',(17.0091979162384,17.3172653529285,-7.32730444150692));
#49489=CARTESIAN_POINT('Ctrl Pts',(16.9458080406878,17.377008133023,-7.33162060424584));
#49490=CARTESIAN_POINT('Ctrl Pts',(16.885663067504,17.4397714478444,-7.33593676698476));
#49491=CARTESIAN_POINT('Ctrl Pts',(16.8274773104956,17.5004902542869,-7.34011233117644));
#49492=CARTESIAN_POINT('Ctrl Pts',(16.7723285700598,17.5640354429535,-7.34428789536812));
#49493=CARTESIAN_POINT('Ctrl Pts',(16.7204869451086,17.6300619310733,-7.3484634595598));
#49494=CARTESIAN_POINT('Ctrl Pts',(16.6660269229228,17.6994232601449,-7.35284992157234));
#49495=CARTESIAN_POINT('Ctrl Pts',(16.6152172172816,17.7715226597539,-7.35723638358488));
#49496=CARTESIAN_POINT('Ctrl Pts',(16.5683186145658,17.845927058072,-7.36162284559743));
#49497=CARTESIAN_POINT('Ctrl Pts',(16.52142001185,17.9203314563902,-7.36600930760997));
#49498=CARTESIAN_POINT('Ctrl Pts',(16.4784327293519,17.9970403100744,-7.37039576962251));
#49499=CARTESIAN_POINT('Ctrl Pts',(16.4395601204679,18.0755945044995,-7.37478223163505));
#49500=CARTESIAN_POINT('Ctrl Pts',(16.399796394139,18.1559494788318,-7.37926924910124));
#49501=CARTESIAN_POINT('Ctrl Pts',(16.3642056179145,18.2385006465143,-7.38375626656742));
#49502=CARTESIAN_POINT('Ctrl Pts',(16.3330179090159,18.3228080169392,-7.3882432840336));
#49503=CARTESIAN_POINT('Ctrl Pts',(16.3019356806123,18.4068302499339,-7.39271512587964));
#49504=CARTESIAN_POINT('Ctrl Pts',(16.2752269677052,18.4925965155752,-7.39718696772568));
#49505=CARTESIAN_POINT('Ctrl Pts',(16.2530742870064,18.5796462112197,-7.40165880957171));
#49506=CARTESIAN_POINT('Ctrl Pts',(16.2309688572624,18.6665102326658,-7.40612111312305));
#49507=CARTESIAN_POINT('Ctrl Pts',(16.2134002030055,18.7546518909164,-7.41058341667439));
#49508=CARTESIAN_POINT('Ctrl Pts',(16.2005019648759,18.8435932689479,-7.41504572022573));
#49509=CARTESIAN_POINT('Ctrl Pts',(16.1876417930138,18.9322721563783,-7.41949485428535));
#49510=CARTESIAN_POINT('Ctrl Pts',(16.1794246278368,19.0217457093711,-7.42394398834497));
#49511=CARTESIAN_POINT('Ctrl Pts',(16.1759333991831,19.1115250494595,-7.42839312240459));
#49512=CARTESIAN_POINT('Ctrl Pts',(16.1746525201579,19.1444637323753,-7.43002544244498));
#49513=CARTESIAN_POINT('Ctrl Pts',(16.1740072831437,19.177443453577,-7.43165776248538));
#49514=CARTESIAN_POINT('Ctrl Pts',(16.1740000613162,19.2104396974995,-7.43329008252577));
#49515=CARTESIAN_POINT('Ctrl Pts',(16.1781030359051,19.2104411453813,-7.4332901097715));
#49516=CARTESIAN_POINT('Ctrl Pts',(16.1790025448085,19.6723916862602,-7.4561794192865));
#49517=CARTESIAN_POINT('Ctrl Pts',(16.519742516428,20.9911304253782,-7.52146066436197));
#49518=CARTESIAN_POINT('Ctrl Pts',(18.3750628632639,22.0833380538217,-7.61589315312154));
#49519=CARTESIAN_POINT('Ctrl Pts',(19.8237022835423,21.5931889594048,-7.68743633236609));
#49520=CARTESIAN_POINT('Ctrl Pts',(20.2923705327634,21.239586948775,-7.71658757605017));
#49521=CARTESIAN_POINT('',(16.1738764730989,19.2121301833587,-7.36670989022851));
#49522=CARTESIAN_POINT('Ctrl Pts',(16.1703788196327,19.2121317274208,-7.36670989022851));
#49523=CARTESIAN_POINT('Ctrl Pts',(16.1700290407744,19.2754624167648,-7.36987218932674));
#49524=CARTESIAN_POINT('Ctrl Pts',(16.2008981366677,20.1874206696652,-7.41542642398544));
#49525=CARTESIAN_POINT('Ctrl Pts',(17.2895132664939,21.8712161675055,-7.50337259420461));
#49526=CARTESIAN_POINT('Ctrl Pts',(19.3719151151867,21.8671174429886,-7.59471149354706));
#49527=CARTESIAN_POINT('Ctrl Pts',(20.1912479901919,21.3237995976637,-7.64365845732902));
#49528=CARTESIAN_POINT('Ctrl Pts',(20.2947700725713,21.2427129721481,-7.65021348555051));
#49529=CARTESIAN_POINT('Ctrl Pts',(20.2935358855687,21.2411349269503,-6.8500446225637));
#49530=CARTESIAN_POINT('Ctrl Pts',(20.3601338969406,21.1899747861817,-6.85422899519217));
#49531=CARTESIAN_POINT('Ctrl Pts',(20.4241220194898,21.1356031650462,-6.85841336782063));
#49532=CARTESIAN_POINT('Ctrl Pts',(20.4851928134884,21.0783306429196,-6.86259774044909));
#49533=CARTESIAN_POINT('Ctrl Pts',(20.5090109309219,21.055993883097,-6.86422968056521));
#49534=CARTESIAN_POINT('Ctrl Pts',(20.5323857243709,21.0332162494999,-6.86586162068134));
#49535=CARTESIAN_POINT('Ctrl Pts',(20.5553006227462,21.0100175211999,-6.86749356079746));
#49536=CARTESIAN_POINT('Ctrl Pts',(20.6140591953844,20.9505311495128,-6.87167819519051));
#49537=CARTESIAN_POINT('Ctrl Pts',(20.6700096812721,20.8880523361676,-6.87586282958356));
#49538=CARTESIAN_POINT('Ctrl Pts',(20.7228319806689,20.8228769657355,-6.8800474639766));
#49539=CARTESIAN_POINT('Ctrl Pts',(20.7755790940605,20.7577943643761,-6.88422614206055));
#49540=CARTESIAN_POINT('Ctrl Pts',(20.8252065780214,20.6900231841701,-6.88840482014449));
#49541=CARTESIAN_POINT('Ctrl Pts',(20.8714311671561,20.6198960237255,-6.89258349822843));
#49542=CARTESIAN_POINT('Ctrl Pts',(20.9184842988301,20.5485118843294,-6.89683707611387));
#49543=CARTESIAN_POINT('Ctrl Pts',(20.9620110031542,20.4746868150558,-6.9010906539993));
#49544=CARTESIAN_POINT('Ctrl Pts',(21.0017554861493,20.3988068256412,-6.90534423188474));
#49545=CARTESIAN_POINT('Ctrl Pts',(21.0407294447865,20.324397917889,-6.90951534586269));
#49546=CARTESIAN_POINT('Ctrl Pts',(21.0760663016048,20.2480134825273,-6.91368645984064));
#49547=CARTESIAN_POINT('Ctrl Pts',(21.1075695674518,20.1700451024153,-6.91785757381859));
#49548=CARTESIAN_POINT('Ctrl Pts',(21.1390622620736,20.0921028853463,-6.92202728813896));
#49549=CARTESIAN_POINT('Ctrl Pts',(21.1667237483346,20.0125782052865,-6.92619700245933));
#49550=CARTESIAN_POINT('Ctrl Pts',(21.1904053024889,19.9318834787289,-6.9303667167797));
#49551=CARTESIAN_POINT('Ctrl Pts',(21.214086013952,19.8511916236359,-6.93453628272375));
#49552=CARTESIAN_POINT('Ctrl Pts',(21.2337869461661,19.7693302464837,-6.93870584866779));
#49553=CARTESIAN_POINT('Ctrl Pts',(21.2494093711531,19.6867264923413,-6.94287541461183));
#49554=CARTESIAN_POINT('Ctrl Pts',(21.2655810613302,19.601218492106,-6.94719157735075));
#49555=CARTESIAN_POINT('Ctrl Pts',(21.2773820094429,19.5149154578639,-6.95150774008968));
#49556=CARTESIAN_POINT('Ctrl Pts',(21.2847607940422,19.4283001877063,-6.9558239028286));
#49557=CARTESIAN_POINT('Ctrl Pts',(21.2918992155093,19.3445064008638,-6.95999946702028));
#49558=CARTESIAN_POINT('Ctrl Pts',(21.2948991834511,19.2604208803107,-6.96417503121195));
#49559=CARTESIAN_POINT('Ctrl Pts',(21.2937672733171,19.1764817953118,-6.96835059540363));
#49560=CARTESIAN_POINT('Ctrl Pts',(21.2925781930931,19.0883031466757,-6.97273705741617));
#49561=CARTESIAN_POINT('Ctrl Pts',(21.2868289009944,19.0002866979193,-6.97712351942871));
#49562=CARTESIAN_POINT('Ctrl Pts',(21.2765884850301,18.9129332360151,-6.98150998144125));
#49563=CARTESIAN_POINT('Ctrl Pts',(21.2663480690658,18.8255797741109,-6.9858964434538));
#49564=CARTESIAN_POINT('Ctrl Pts',(21.2516167014297,18.7388898583324,-6.99028290546634));
#49565=CARTESIAN_POINT('Ctrl Pts',(21.2325245180282,18.6533484665025,-6.99466936747888));
#49566=CARTESIAN_POINT('Ctrl Pts',(21.2143107942864,18.5717429609135,-6.99885400187193));
#49567=CARTESIAN_POINT('Ctrl Pts',(21.1920609365757,18.490878859979,-7.00303863626498));
#49568=CARTESIAN_POINT('Ctrl Pts',(21.1658504730776,18.4111854736302,-7.00722327065802));
#49569=CARTESIAN_POINT('Ctrl Pts',(21.1396773169301,18.3316055209528,-7.01140194874197));
#49570=CARTESIAN_POINT('Ctrl Pts',(21.109554895207,18.2531934061979,-7.01558062682591));
#49571=CARTESIAN_POINT('Ctrl Pts',(21.0756095445168,18.1763673400535,-7.01975930490986));
#49572=CARTESIAN_POINT('Ctrl Pts',(21.0410557478115,18.0981642218874,-7.02401288279529));
#49573=CARTESIAN_POINT('Ctrl Pts',(21.0025407271243,18.0216050420064,-7.02826646068073));
#49574=CARTESIAN_POINT('Ctrl Pts',(20.9602505991268,17.9471138224161,-7.03252003856616));
#49575=CARTESIAN_POINT('Ctrl Pts',(20.9187803477829,17.8740667604752,-7.03669115254411));
#49576=CARTESIAN_POINT('Ctrl Pts',(20.8736802961219,17.8030086099539,-7.04086226652207));
#49577=CARTESIAN_POINT('Ctrl Pts',(20.8251733475076,17.7343165435092,-7.04503338050002));
#49578=CARTESIAN_POINT('Ctrl Pts',(20.7766826758684,17.6656475273507,-7.04920309482039));
#49579=CARTESIAN_POINT('Ctrl Pts',(20.7247876428631,17.5993433939188,-7.05337280914077));
#49580=CARTESIAN_POINT('Ctrl Pts',(20.669754524153,17.5357524295731,-7.05754252346114));
#49581=CARTESIAN_POINT('Ctrl Pts',(20.6147233637575,17.4721637280668,-7.06171208940518));
#49582=CARTESIAN_POINT('Ctrl Pts',(20.556554641366,17.4112883509861,-7.06588165534923));
#49583=CARTESIAN_POINT('Ctrl Pts',(20.4955540788025,17.3534405184613,-7.07005122129327));
#49584=CARTESIAN_POINT('Ctrl Pts',(20.4324088117115,17.2935588275079,-7.07436738403219));
#49585=CARTESIAN_POINT('Ctrl Pts',(20.3662292470559,17.2369219021169,-7.07868354677111));
#49586=CARTESIAN_POINT('Ctrl Pts',(20.2973935081709,17.1838343090391,-7.08299970951003));
#49587=CARTESIAN_POINT('Ctrl Pts',(20.2308000862399,17.132476038722,-7.08717527370171));
#49588=CARTESIAN_POINT('Ctrl Pts',(20.1617212960249,17.0844396429708,-7.09135083789339));
#49589=CARTESIAN_POINT('Ctrl Pts',(20.0905291277018,17.0399567655856,-7.09552640208507));
#49590=CARTESIAN_POINT('Ctrl Pts',(20.0157412122,16.9932271638116,-7.09991286409762));
#49591=CARTESIAN_POINT('Ctrl Pts',(19.9386213249318,16.9504197742736,-7.10429932611015));
#49592=CARTESIAN_POINT('Ctrl Pts',(19.8596279445188,16.9117475713792,-7.10868578812269));
#49593=CARTESIAN_POINT('Ctrl Pts',(19.7806345641058,16.8730753684849,-7.11307225013523));
#49594=CARTESIAN_POINT('Ctrl Pts',(19.6997682540137,16.8385385101708,-7.11745871214778));
#49595=CARTESIAN_POINT('Ctrl Pts',(19.6175072439402,16.8082900820313,-7.12184517416032));
#49596=CARTESIAN_POINT('Ctrl Pts',(19.5390311848803,16.7794334289094,-7.12602980855336));
#49597=CARTESIAN_POINT('Ctrl Pts',(19.4589938470389,16.7543718340009,-7.13021444294641));
#49598=CARTESIAN_POINT('Ctrl Pts',(19.3777970941006,16.733274167381,-7.13439907733946));
#49599=CARTESIAN_POINT('Ctrl Pts',(19.2967159146901,16.7122065306782,-7.1385777554234));
#49600=CARTESIAN_POINT('Ctrl Pts',(19.2144790396056,16.6950917298573,-7.14275643350734));
#49601=CARTESIAN_POINT('Ctrl Pts',(19.1315065014626,16.6820499053372,-7.14693511159128));
#49602=CARTESIAN_POINT('Ctrl Pts',(19.0470467402047,16.6687743154856,-7.15118868947672));
#49603=CARTESIAN_POINT('Ctrl Pts',(18.9618251354749,16.6597193207395,-7.15544226736216));
#49604=CARTESIAN_POINT('Ctrl Pts',(18.8762989641012,16.654957941501,-7.15969584524759));
#49605=CARTESIAN_POINT('Ctrl Pts',(18.7924308844501,16.6502888708901,-7.16386695922554));
#49606=CARTESIAN_POINT('Ctrl Pts',(18.7082704224839,16.6497484479464,-7.1680380732035));
#49607=CARTESIAN_POINT('Ctrl Pts',(18.6242553740812,16.6533534026215,-7.17220918718145));
#49608=CARTESIAN_POINT('Ctrl Pts',(18.5402685177394,16.6569571476192,-7.17637890150182));
#49609=CARTESIAN_POINT('Ctrl Pts',(18.4564274372811,16.6647034879404,-7.18054861582219));
#49610=CARTESIAN_POINT('Ctrl Pts',(18.3731691163825,16.6765570486934,-7.18471833014257));
#49611=CARTESIAN_POINT('Ctrl Pts',(18.2899137581723,16.6884101876458,-7.18888789608661));
#49612=CARTESIAN_POINT('Ctrl Pts',(18.2072415736113,16.7043701907562,-7.19305746203065));
#49613=CARTESIAN_POINT('Ctrl Pts',(18.1255822535274,16.7243500757491,-7.1972270279747));
#49614=CARTESIAN_POINT('Ctrl Pts',(18.041051892487,16.7450324288504,-7.20154319071362));
#49615=CARTESIAN_POINT('Ctrl Pts',(17.9576074580676,16.7700224760727,-7.20585935345254));
#49616=CARTESIAN_POINT('Ctrl Pts',(17.8757097136975,16.7991671317359,-7.21017551619146));
#49617=CARTESIAN_POINT('Ctrl Pts',(17.7964797797362,16.8273624033065,-7.21435108038314));
#49618=CARTESIAN_POINT('Ctrl Pts',(17.7186977338734,16.8594455439839,-7.21852664457482));
#49619=CARTESIAN_POINT('Ctrl Pts',(17.6427597031133,16.8952291532946,-7.2227022087665));
#49620=CARTESIAN_POINT('Ctrl Pts',(17.5629862229451,16.9328201076441,-7.22708867077904));
#49621=CARTESIAN_POINT('Ctrl Pts',(17.4852484504759,16.9744949002993,-7.23147513279159));
#49622=CARTESIAN_POINT('Ctrl Pts',(17.409973629261,17.0199833023029,-7.23586159480413));
#49623=CARTESIAN_POINT('Ctrl Pts',(17.3346988080461,17.0654717043064,-7.24024805681667));
#49624=CARTESIAN_POINT('Ctrl Pts',(17.2618873758783,17.1147733273606,-7.24463451882921));
#49625=CARTESIAN_POINT('Ctrl Pts',(17.1919269101811,17.1675689183003,-7.24902098084175));
#49626=CARTESIAN_POINT('Ctrl Pts',(17.1258771580207,17.2174132934338,-7.25316224442401));
#49627=CARTESIAN_POINT('Ctrl Pts',(17.0621112325389,17.2705657001619,-7.25730350800627));
#49628=CARTESIAN_POINT('Ctrl Pts',(17.0009846311416,17.326787238314,-7.26144477158852));
#49629=CARTESIAN_POINT('Ctrl Pts',(16.9399453026366,17.3829285067285,-7.26558012252321));
#49630=CARTESIAN_POINT('Ctrl Pts',(16.8815381604268,17.4421298917806,-7.2697154734579));
#49631=CARTESIAN_POINT('Ctrl Pts',(16.8260879518441,17.5041105435613,-7.27385082439259));
#49632=CARTESIAN_POINT('Ctrl Pts',(16.7707013118209,17.5660201402305,-7.27798143452813));
#49633=CARTESIAN_POINT('Ctrl Pts',(16.7182651826551,17.6307023247235,-7.28211204466367));
#49634=CARTESIAN_POINT('Ctrl Pts',(16.6690684130045,17.6978385608177,-7.28624265479921));
#49635=CARTESIAN_POINT('Ctrl Pts',(16.6199019406792,17.7649334517505,-7.29037072114092));
#49636=CARTESIAN_POINT('Ctrl Pts',(16.5739711466916,17.8344790168686,-7.29449878748264));
#49637=CARTESIAN_POINT('Ctrl Pts',(16.5315246255303,17.9061236744984,-7.29862685382436));
#49638=CARTESIAN_POINT('Ctrl Pts',(16.4890908665707,17.977746791056,-7.3027536789992));
#49639=CARTESIAN_POINT('Ctrl Pts',(16.4501395400176,18.0514673424197,-7.30688050417405));
#49640=CARTESIAN_POINT('Ctrl Pts',(16.4148750854129,18.1269060785424,-7.3110073293489));
#49641=CARTESIAN_POINT('Ctrl Pts',(16.3796101195078,18.2023459084537,-7.31513421435872));
#49642=CARTESIAN_POINT('Ctrl Pts',(16.3480323287909,18.2795035453344,-7.31926109936854));
#49643=CARTESIAN_POINT('Ctrl Pts',(16.3202988339461,18.3579779129531,-7.32338798437835));
#49644=CARTESIAN_POINT('Ctrl Pts',(16.2925397363851,18.4365247257132,-7.32751867920247));
#49645=CARTESIAN_POINT('Ctrl Pts',(16.2686321752694,18.516390251046,-7.33164937402659));
#49646=CARTESIAN_POINT('Ctrl Pts',(16.2486837569799,18.5971570459957,-7.33578006885071));
#49647=CARTESIAN_POINT('Ctrl Pts',(16.2287250388403,18.6779655427923,-7.33991289645232));
#49648=CARTESIAN_POINT('Ctrl Pts',(16.2127296214478,18.7596757735077,-7.34404572405394));
#49649=CARTESIAN_POINT('Ctrl Pts',(16.2007537416511,18.8418612800569,-7.34817855165556));
#49650=CARTESIAN_POINT('Ctrl Pts',(16.1887593096482,18.9241741027186,-7.35231778154836));
#49651=CARTESIAN_POINT('Ctrl Pts',(16.180796886798,19.0069632027562,-7.35645701144116));
#49652=CARTESIAN_POINT('Ctrl Pts',(16.176870697397,19.0897988045885,-7.36059624133397));
#49653=CARTESIAN_POINT('Ctrl Pts',(16.1749377014765,19.1305815748691,-7.36263412429881));
#49654=CARTESIAN_POINT('Ctrl Pts',(16.1739822581149,19.1713756409971,-7.36467200726366));
#49655=CARTESIAN_POINT('Ctrl Pts',(16.1740002494514,19.2121301287168,-7.36670989022851));
#49656=CARTESIAN_POINT('Origin',(18.734,19.211,1.76670989022852));
#49657=CARTESIAN_POINT('',(20.2935358855687,21.2411349269503,-6.05008448348788));
#49658=CARTESIAN_POINT('',(20.2954006757859,21.2435252751206,-6.11677130154247));
#49659=CARTESIAN_POINT('',(20.2935358855687,21.2411349269503,1.76670989022852));
#49660=CARTESIAN_POINT('',(16.1740008768645,19.208881145288,-6.6332901097715));
#49661=CARTESIAN_POINT('Ctrl Pts',(20.2954006757859,21.2435252751206,-6.11677130154247));
#49662=CARTESIAN_POINT('Ctrl Pts',(20.8926533935168,20.777292913641,-6.1545808581957));
#49663=CARTESIAN_POINT('Ctrl Pts',(21.7124083704566,19.1915607510674,-6.23478235040939));
#49664=CARTESIAN_POINT('Ctrl Pts',(20.433793589474,16.7062061261689,-6.35737577818358));
#49665=CARTESIAN_POINT('Ctrl Pts',(17.5479307751794,16.4259451726882,-6.48455158486501));
#49666=CARTESIAN_POINT('Ctrl Pts',(16.2478508564243,18.0710820233979,-6.57652302872766));
#49667=CARTESIAN_POINT('Ctrl Pts',(16.1710772436132,19.0646440698247,-6.62610253702982));
#49668=CARTESIAN_POINT('Ctrl Pts',(16.172362658312,19.2088797893707,-6.6332901097715));
#49669=CARTESIAN_POINT('Ctrl Pts',(16.1740008768645,19.208881145288,-6.6332901097715));
#49670=CARTESIAN_POINT('Ctrl Pts',(16.1739325519701,19.291431245901,-6.63740642252224));
#49671=CARTESIAN_POINT('Ctrl Pts',(16.1778613169669,19.3741241408158,-6.64152273527298));
#49672=CARTESIAN_POINT('Ctrl Pts',(16.1858020059738,19.456534077555,-6.64563904802372));
#49673=CARTESIAN_POINT('Ctrl Pts',(16.1937337220434,19.5388508914938,-6.64975070936243));
#49674=CARTESIAN_POINT('Ctrl Pts',(16.2056683130375,19.6208849121504,-6.65386237070114));
#49675=CARTESIAN_POINT('Ctrl Pts',(16.2215685692311,19.7022110602219,-6.65797403203985));
#49676=CARTESIAN_POINT('Ctrl Pts',(16.2374592000151,19.7834879765409,-6.66208320433539));
#49677=CARTESIAN_POINT('Ctrl Pts',(16.2573106430752,19.8640574053625,-6.66619237663093));
#49678=CARTESIAN_POINT('Ctrl Pts',(16.2810340922892,19.9435013690146,-6.67030154892647));
#49679=CARTESIAN_POINT('Ctrl Pts',(16.3047507902537,20.0229227244023,-6.67440955182852));
#49680=CARTESIAN_POINT('Ctrl Pts',(16.3323371713261,20.1012187954775,-6.67851755473057));
#49681=CARTESIAN_POINT('Ctrl Pts',(16.3636541468012,20.1779852823199,-6.68262555763262));
#49682=CARTESIAN_POINT('Ctrl Pts',(16.3949722554066,20.2547545467753,-6.68673370917299));
#49683=CARTESIAN_POINT('Ctrl Pts',(16.4300210447236,20.3299936782016,-6.69084186071336));
#49684=CARTESIAN_POINT('Ctrl Pts',(16.4686133150906,20.4033184003592,-6.69495001225373));
#49685=CARTESIAN_POINT('Ctrl Pts',(16.5072438266208,20.4767157801408,-6.69906223457025));
#49686=CARTESIAN_POINT('Ctrl Pts',(16.5494246053548,20.5481945435127,-6.70317445688677));
#49687=CARTESIAN_POINT('Ctrl Pts',(16.5949228757402,20.6173957680782,-6.70728667920329));
#49688=CARTESIAN_POINT('Ctrl Pts',(16.6404458510681,20.6866345679682,-6.71140113440064));
#49689=CARTESIAN_POINT('Ctrl Pts',(16.6892896206456,20.7535929860938,-6.715515589598));
#49690=CARTESIAN_POINT('Ctrl Pts',(16.7411800554792,20.8179438909682,-6.71963004479535));
#49691=CARTESIAN_POINT('Ctrl Pts',(16.7931561866085,20.8824010704228,-6.7237512949554));
#49692=CARTESIAN_POINT('Ctrl Pts',(16.8481887081045,20.9442417891331,-6.72787254511546));
#49693=CARTESIAN_POINT('Ctrl Pts',(16.9059658904508,21.0031750177716,-6.73199379527552));
#49694=CARTESIAN_POINT('Ctrl Pts',(16.9382542996129,21.0361094760171,-6.73429692959297));
#49695=CARTESIAN_POINT('Ctrl Pts',(16.9713992632832,21.068136611825,-6.73660006391043));
#49696=CARTESIAN_POINT('Ctrl Pts',(17.0053421035809,21.0992112903877,-6.73890319822789));
#49697=CARTESIAN_POINT('Ctrl Pts',(17.067013876621,21.1556718136325,-6.74308783262094));
#49698=CARTESIAN_POINT('Ctrl Pts',(17.1315694533286,21.2092127933028,-6.74727246701399));
#49699=CARTESIAN_POINT('Ctrl Pts',(17.198701023428,21.259525580152,-6.75145710140704));
#49700=CARTESIAN_POINT('Ctrl Pts',(17.2657370400465,21.3097667529765,-6.75563577949099));
#49701=CARTESIAN_POINT('Ctrl Pts',(17.3353414020479,21.3567885864286,-6.75981445757493));
#49702=CARTESIAN_POINT('Ctrl Pts',(17.4071710083241,21.4003206313485,-6.76399313565888));
#49703=CARTESIAN_POINT('Ctrl Pts',(17.4802881086698,21.4446329568877,-6.76824671354431));
#49704=CARTESIAN_POINT('Ctrl Pts',(17.5557106573433,21.4853288288424,-6.77250029142975));
#49705=CARTESIAN_POINT('Ctrl Pts',(17.6330432222703,21.5221672751169,-6.77675386931518));
#49706=CARTESIAN_POINT('Ctrl Pts',(17.7088765445241,21.5582915362259,-6.78092498329313));
#49707=CARTESIAN_POINT('Ctrl Pts',(17.7865460506904,21.5907063974352,-6.78509609727109));
#49708=CARTESIAN_POINT('Ctrl Pts',(17.8656529884827,21.6192303601585,-6.78926721124904));
#49709=CARTESIAN_POINT('Ctrl Pts',(17.9447333811781,21.6477447513906,-6.79343692556941));
#49710=CARTESIAN_POINT('Ctrl Pts',(18.0252498151568,21.6723706812234,-6.79760663988978));
#49711=CARTESIAN_POINT('Ctrl Pts',(18.1067845307988,21.6929751721552,-6.80177635421016));
#49712=CARTESIAN_POINT('Ctrl Pts',(18.1883163450855,21.7135789298907,-6.80594592015419));
#49713=CARTESIAN_POINT('Ctrl Pts',(18.2708659227708,21.7301614213603,-6.81011548609823));
#49714=CARTESIAN_POINT('Ctrl Pts',(18.3540026821446,21.7426401873929,-6.81428505204227));
#49715=CARTESIAN_POINT('Ctrl Pts',(18.4400624274178,21.755557691445,-6.81860121478119));
#49716=CARTESIAN_POINT('Ctrl Pts',(18.5267508916658,21.7640774486062,-6.82291737752011));
#49717=CARTESIAN_POINT('Ctrl Pts',(18.6135836740995,21.7681663826307,-6.82723354025903));
#49718=CARTESIAN_POINT('Ctrl Pts',(18.6975878877785,21.7721221200595,-6.83140910445071));
#49719=CARTESIAN_POINT('Ctrl Pts',(18.7817266907697,21.7719313177434,-6.83558466864238));
#49720=CARTESIAN_POINT('Ctrl Pts',(18.8655624783152,21.7676171622477,-6.83976023283406));
#49721=CARTESIAN_POINT('Ctrl Pts',(18.953632612189,21.7630851090138,-6.8441466948466));
#49722=CARTESIAN_POINT('Ctrl Pts',(19.0413677347562,21.7540022746857,-6.84853315685915));
#49723=CARTESIAN_POINT('Ctrl Pts',(19.1282700391325,21.7404566879554,-6.85291961887169));
#49724=CARTESIAN_POINT('Ctrl Pts',(19.2151723435088,21.7269111012252,-6.85730608088423));
#49725=CARTESIAN_POINT('Ctrl Pts',(19.3012412773526,21.7089029553709,-6.86169254289678));
#49726=CARTESIAN_POINT('Ctrl Pts',(19.3859971465595,21.6865806835727,-6.86607900490932));
#49727=CARTESIAN_POINT('Ctrl Pts',(19.4675566076895,21.6651002542397,-6.87030003976341));
#49728=CARTESIAN_POINT('Ctrl Pts',(19.5482065108308,21.6395446517759,-6.87452107461749));
#49729=CARTESIAN_POINT('Ctrl Pts',(19.6275095396711,21.6100082747912,-6.87874210947158));
#49730=CARTESIAN_POINT('Ctrl Pts',(19.7060066089446,21.5807720770802,-6.8829202457949));
#49731=CARTESIAN_POINT('Ctrl Pts',(19.7831836018448,21.5476357741988,-6.88709838211823));
#49732=CARTESIAN_POINT('Ctrl Pts',(19.8586276861513,21.5107418480217,-6.89127651844155));
#49733=CARTESIAN_POINT('Ctrl Pts',(19.9352336905536,21.4732797156739,-6.89551900256102));
#49734=CARTESIAN_POINT('Ctrl Pts',(20.0100524876427,21.4319433469969,-6.89976148668049));
#49735=CARTESIAN_POINT('Ctrl Pts',(20.0826708300222,21.3869335909552,-6.90400397079996));
#49736=CARTESIAN_POINT('Ctrl Pts',(20.1552891724016,21.3419238349136,-6.90824645491943));
#49737=CARTESIAN_POINT('Ctrl Pts',(20.2257066125816,21.2932409145431,-6.9124889390389));
#49738=CARTESIAN_POINT('Ctrl Pts',(20.2935358855687,21.2411349269503,-6.91673142315837));
#49739=CARTESIAN_POINT('',(16.174000571626,19.2127107672549,-6.56670989025839));
#49740=CARTESIAN_POINT('Ctrl Pts',(16.174000571626,19.2127107672549,-6.56670989025838));
#49741=CARTESIAN_POINT('Ctrl Pts',(16.1740643617891,19.3081666398866,-6.57143929947811));
#49742=CARTESIAN_POINT('Ctrl Pts',(16.1794711562484,19.4034153336876,-6.57616870869783));
#49743=CARTESIAN_POINT('Ctrl Pts',(16.1901275024527,19.4979019278825,-6.58089811791755));
#49744=CARTESIAN_POINT('Ctrl Pts',(16.200836414009,19.5928546031322,-6.58565085624608));
#49745=CARTESIAN_POINT('Ctrl Pts',(16.2168466650982,19.6870374428256,-6.59040359457461));
#49746=CARTESIAN_POINT('Ctrl Pts',(16.2380139506883,19.7799056526714,-6.59515633290315));
#49747=CARTESIAN_POINT('Ctrl Pts',(16.2593038089226,19.8733116311407,-6.59993659274364));
#49748=CARTESIAN_POINT('Ctrl Pts',(16.2858104835354,19.9653875176628,-6.60471685258415));
#49749=CARTESIAN_POINT('Ctrl Pts',(16.3173390825683,20.0556005032904,-6.60949711242465));
#49750=CARTESIAN_POINT('Ctrl Pts',(16.3253523527952,20.0785289255476,-6.61071205742796));
#49751=CARTESIAN_POINT('Ctrl Pts',(16.3336897868424,20.101337126465,-6.61192700243127));
#49752=CARTESIAN_POINT('Ctrl Pts',(16.3423477078173,20.1240166007785,-6.61314194743458));
#49753=CARTESIAN_POINT('Ctrl Pts',(16.3721681801721,20.2021315014283,-6.61732658182763));
#49754=CARTESIAN_POINT('Ctrl Pts',(16.405875193857,20.2789292632221,-6.62151121622068));
#49755=CARTESIAN_POINT('Ctrl Pts',(16.4433319467771,20.3539960060927,-6.62569585061372));
#49756=CARTESIAN_POINT('Ctrl Pts',(16.4807353846457,20.4289559007464,-6.62987452869767));
#49757=CARTESIAN_POINT('Ctrl Pts',(16.5218777565726,20.5021892624269,-6.63405320678162));
#49758=CARTESIAN_POINT('Ctrl Pts',(16.5665735905077,20.5733005393214,-6.63823188486556));
#49759=CARTESIAN_POINT('Ctrl Pts',(16.6120705651437,20.6456864347474,-6.642485462751));
#49760=CARTESIAN_POINT('Ctrl Pts',(16.6612494744651,20.715872969927,-6.64673904063643));
#49761=CARTESIAN_POINT('Ctrl Pts',(16.7138648542456,20.7834674854787,-6.65099261852187));
#49762=CARTESIAN_POINT('Ctrl Pts',(16.7654601822185,20.8497515494465,-6.65516373249982));
#49763=CARTESIAN_POINT('Ctrl Pts',(16.8203596287513,20.9135428198972,-6.65933484647778));
#49764=CARTESIAN_POINT('Ctrl Pts',(16.8782881026494,20.9745003130228,-6.66350596045573));
#49765=CARTESIAN_POINT('Ctrl Pts',(16.9361971380886,21.0354373512729,-6.6676756747761));
#49766=CARTESIAN_POINT('Ctrl Pts',(16.9971328656302,21.0935421675084,-6.67184538909648));
#49767=CARTESIAN_POINT('Ctrl Pts',(17.0607814536892,21.1485086312792,-6.67601510341685));
#49768=CARTESIAN_POINT('Ctrl Pts',(17.1244277768583,21.2034731391074,-6.68018466936089));
#49769=CARTESIAN_POINT('Ctrl Pts',(17.1907864198801,21.2552992164785,-6.68435423530494));
#49770=CARTESIAN_POINT('Ctrl Pts',(17.2595094445544,21.3037201441907,-6.68852380124898));
#49771=CARTESIAN_POINT('Ctrl Pts',(17.3306486859971,21.3538434919877,-6.6928399639879));
#49772=CARTESIAN_POINT('Ctrl Pts',(17.404321234744,21.4003174810233,-6.69715612672682));
#49773=CARTESIAN_POINT('Ctrl Pts',(17.4801089073794,21.4428954114937,-6.70147228946574));
#49774=CARTESIAN_POINT('Ctrl Pts',(17.5534278045501,21.4840863703575,-6.70564785365742));
#49775=CARTESIAN_POINT('Ctrl Pts',(17.6287256988458,21.5216310329473,-6.7098234178491));
#49776=CARTESIAN_POINT('Ctrl Pts',(17.7056010183995,21.555353969571,-6.71399898204078));
#49777=CARTESIAN_POINT('Ctrl Pts',(17.7863591275902,21.5907801715548,-6.71838544405332));
#49778=CARTESIAN_POINT('Ctrl Pts',(17.8688576552588,21.6219882241026,-6.72277190606586));
#49779=CARTESIAN_POINT('Ctrl Pts',(17.9526121488768,21.6488336748263,-6.7271583680784));
#49780=CARTESIAN_POINT('Ctrl Pts',(18.0363666424948,21.67567912555,-6.73154483009094));
#49781=CARTESIAN_POINT('Ctrl Pts',(18.1213765216826,21.6981618996353,-6.73593129210348));
#49782=CARTESIAN_POINT('Ctrl Pts',(18.20714644876,21.7161996598167,-6.74031775411602));
#49783=CARTESIAN_POINT('Ctrl Pts',(18.2889778682176,21.7334091360257,-6.7445027922187));
#49784=CARTESIAN_POINT('Ctrl Pts',(18.3718056859211,21.7466369348047,-6.74868783032139));
#49785=CARTESIAN_POINT('Ctrl Pts',(18.4552077229433,21.7557740304894,-6.75287286842408));
#49786=CARTESIAN_POINT('Ctrl Pts',(18.5384664989634,21.76489543124,-6.75705071782042));
#49787=CARTESIAN_POINT('Ctrl Pts',(18.6222970795584,21.7699400516429,-6.76122856721677));
#49788=CARTESIAN_POINT('Ctrl Pts',(18.7062667332565,21.7708497740914,-6.76540641661311));
#49789=CARTESIAN_POINT('Ctrl Pts',(18.7901543122251,21.771758607347,-6.76958018244065));
#49790=CARTESIAN_POINT('Ctrl Pts',(18.8741802371502,21.7685405617463,-6.77375394826818));
#49791=CARTESIAN_POINT('Ctrl Pts',(18.9579070743406,21.7611893306302,-6.77792771409572));
#49792=CARTESIAN_POINT('Ctrl Pts',(19.0415771929613,21.7538430794146,-6.78209865251408));
#49793=CARTESIAN_POINT('Ctrl Pts',(19.1249481693622,21.7423692437104,-6.78626959093244));
#49794=CARTESIAN_POINT('Ctrl Pts',(19.2075843584856,21.7268135573603,-6.7904405293508));
#49795=CARTESIAN_POINT('Ctrl Pts',(19.2901893576106,21.7112637423098,-6.7946098935005));
#49796=CARTESIAN_POINT('Ctrl Pts',(19.3720596691157,21.691635223593,-6.79877925765021));
#49797=CARTESIAN_POINT('Ctrl Pts',(19.4527679051965,21.6680251725327,-6.80294862179992));
#49798=CARTESIAN_POINT('Ctrl Pts',(19.5335042821167,21.6444068892686,-6.80711943969725));
#49799=CARTESIAN_POINT('Ctrl Pts',(19.6130773298807,21.61680442152,-6.81129025759458));
#49800=CARTESIAN_POINT('Ctrl Pts',(19.6910737323164,21.585365151132,-6.81546107549191));
#49801=CARTESIAN_POINT('Ctrl Pts',(19.769082010496,21.5539210937959,-6.81963252843861));
#49802=CARTESIAN_POINT('Ctrl Pts',(19.8455127429604,21.5186392539808,-6.8238039813853));
#49803=CARTESIAN_POINT('Ctrl Pts',(19.9199734317163,21.4797148386836,-6.827975434332));
#49804=CARTESIAN_POINT('Ctrl Pts',(19.9945177108365,21.4407467264221,-6.83215157019631));
#49805=CARTESIAN_POINT('Ctrl Pts',(20.0670871265665,21.3981280958129,-6.83632770606063));
#49806=CARTESIAN_POINT('Ctrl Pts',(20.1373150369655,21.3520994621985,-6.84050384192494));
#49807=CARTESIAN_POINT('Ctrl Pts',(20.19079582316,21.3170471945292,-6.84368410213786));
#49808=CARTESIAN_POINT('Ctrl Pts',(20.2429192162059,21.2800183091488,-6.84686436235078));
#49809=CARTESIAN_POINT('Ctrl Pts',(20.2935358855687,21.2411349269503,-6.8500446225637));
#49810=CARTESIAN_POINT('Ctrl Pts',(20.2935358855687,21.2411349269503,-6.05008448348788));
#49811=CARTESIAN_POINT('Ctrl Pts',(20.3602243251599,21.1899053198368,-6.05425482437397));
#49812=CARTESIAN_POINT('Ctrl Pts',(20.4243678378452,21.1354001087936,-6.05842516526005));
#49813=CARTESIAN_POINT('Ctrl Pts',(20.4856397822034,21.0779113726695,-6.06259550614614));
#49814=CARTESIAN_POINT('Ctrl Pts',(20.5469803588776,21.0203582419002,-6.06677051834071));
#49815=CARTESIAN_POINT('Ctrl Pts',(20.6054426129598,20.9598152326617,-6.07094553053529));
#49816=CARTESIAN_POINT('Ctrl Pts',(20.6607367282526,20.8966113371719,-6.07512054272987));
#49817=CARTESIAN_POINT('Ctrl Pts',(20.7160670495591,20.8333660564264,-6.07929828867916));
#49818=CARTESIAN_POINT('Ctrl Pts',(20.768224818516,20.7674567823383,-6.08347603462846));
#49819=CARTESIAN_POINT('Ctrl Pts',(20.8169619650072,20.6992437476211,-6.08765378057776));
#49820=CARTESIAN_POINT('Ctrl Pts',(20.8657776938873,20.6309207281468,-6.0918382626058));
#49821=CARTESIAN_POINT('Ctrl Pts',(20.9111615468503,20.5602869221389,-6.09602274463385));
#49822=CARTESIAN_POINT('Ctrl Pts',(20.9529102907763,20.4877290712938,-6.1002072266619));
#49823=CARTESIAN_POINT('Ctrl Pts',(20.9669828856803,20.4632713955407,-6.10161772467755));
#49824=CARTESIAN_POINT('Ctrl Pts',(20.9806428526884,20.4385952862944,-6.1030282226932));
#49825=CARTESIAN_POINT('Ctrl Pts',(20.9938836431733,20.4137160593082,-6.10443872070885));
#49826=CARTESIAN_POINT('Ctrl Pts',(21.0331661282527,20.3399049175952,-6.1086233551019));
#49827=CARTESIAN_POINT('Ctrl Pts',(21.0689017421373,20.2640298565515,-6.11280798949495));
#49828=CARTESIAN_POINT('Ctrl Pts',(21.1008684225543,20.1864659759907,-6.116992623888));
#49829=CARTESIAN_POINT('Ctrl Pts',(21.1327896023584,20.1090124980134,-6.12117130197194));
#49830=CARTESIAN_POINT('Ctrl Pts',(21.1609523307067,20.0298753969622,-6.12534998005589));
#49831=CARTESIAN_POINT('Ctrl Pts',(21.1851803441784,19.9494544131587,-6.12952865813984));
#49832=CARTESIAN_POINT('Ctrl Pts',(21.2098426273792,19.867591941018,-6.13378223602527));
#49833=CARTESIAN_POINT('Ctrl Pts',(21.2304275222058,19.7843995318237,-6.13803581391071));
#49834=CARTESIAN_POINT('Ctrl Pts',(21.2468003698023,19.7003202443405,-6.14228939179614));
#49835=CARTESIAN_POINT('Ctrl Pts',(21.2628557977992,19.6178709979124,-6.14646050577409));
#49836=CARTESIAN_POINT('Ctrl Pts',(21.2748609466779,19.5345694264043,-6.15063161975204));
#49837=CARTESIAN_POINT('Ctrl Pts',(21.2827395777799,19.4508469609111,-6.15480273372999));
#49838=CARTESIAN_POINT('Ctrl Pts',(21.2906155651312,19.3671525892997,-6.15897244805036));
#49839=CARTESIAN_POINT('Ctrl Pts',(21.2943677416632,19.2830380618264,-6.16314216237074));
#49840=CARTESIAN_POINT('Ctrl Pts',(21.2939715980996,19.1989411060454,-6.16731187669111));
#49841=CARTESIAN_POINT('Ctrl Pts',(21.2935754686325,19.1148471427948,-6.17148144263515));
#49842=CARTESIAN_POINT('Ctrl Pts',(21.2890313155854,19.0307712100169,-6.1756510085792));
#49843=CARTESIAN_POINT('Ctrl Pts',(21.2803667494581,18.9471508437493,-6.17982057452325));
#49844=CARTESIAN_POINT('Ctrl Pts',(21.2713975478746,18.8605904885607,-6.18413673726217));
#49845=CARTESIAN_POINT('Ctrl Pts',(21.2580128490967,18.7745188559842,-6.18845290000109));
#49846=CARTESIAN_POINT('Ctrl Pts',(21.2403015155518,18.6894132736133,-6.19276906274001));
#49847=CARTESIAN_POINT('Ctrl Pts',(21.2231671268342,18.6070799966365,-6.19694462693169));
#49848=CARTESIAN_POINT('Ctrl Pts',(21.2019838191122,18.5256512422048,-6.20112019112337));
#49849=CARTESIAN_POINT('Ctrl Pts',(21.1768832583851,18.4455449811374,-6.20529575531505));
#49850=CARTESIAN_POINT('Ctrl Pts',(21.1505149280065,18.361392743258,-6.20968221732759));
#49851=CARTESIAN_POINT('Ctrl Pts',(21.1198234271564,18.278700655445,-6.21406867934013));
#49852=CARTESIAN_POINT('Ctrl Pts',(21.0850182368018,18.197928802983,-6.21845514135267));
#49853=CARTESIAN_POINT('Ctrl Pts',(21.0502130464472,18.117156950521,-6.2228416033652));
#49854=CARTESIAN_POINT('Ctrl Pts',(21.0112944915984,18.0383058200371,-6.22722806537774));
#49855=CARTESIAN_POINT('Ctrl Pts',(20.9685260259017,17.9618028820206,-6.23161452739028));
#49856=CARTESIAN_POINT('Ctrl Pts',(20.9277254007097,17.8888199575867,-6.23579916178333));
#49857=CARTESIAN_POINT('Ctrl Pts',(20.8832694918769,17.8177022301347,-6.23998379617638));
#49858=CARTESIAN_POINT('Ctrl Pts',(20.8353535008892,17.7488394533087,-6.24416843056942));
#49859=CARTESIAN_POINT('Ctrl Pts',(20.7875057123838,17.680074694122,-6.24834710865336));
#49860=CARTESIAN_POINT('Ctrl Pts',(20.7362078848241,17.6135588845842,-6.25252578673731));
#49861=CARTESIAN_POINT('Ctrl Pts',(20.6817007285136,17.5496566061926,-6.25670446482125));
#49862=CARTESIAN_POINT('Ctrl Pts',(20.6262165705999,17.4846089253865,-6.26095804270669));
#49863=CARTESIAN_POINT('Ctrl Pts',(20.5674071330978,17.4222698132395,-6.26521162059212));
#49864=CARTESIAN_POINT('Ctrl Pts',(20.5055720700286,17.3629923158453,-6.26946519847756));
#49865=CARTESIAN_POINT('Ctrl Pts',(20.4449358003181,17.3048640284086,-6.27363631245551));
#49866=CARTESIAN_POINT('Ctrl Pts',(20.3813905208317,17.2496800373396,-6.27780742643346));
#49867=CARTESIAN_POINT('Ctrl Pts',(20.3152577303047,17.1977379727538,-6.28197854041141));
#49868=CARTESIAN_POINT('Ctrl Pts',(20.2491471312743,17.1458133378293,-6.28614825473179));
#49869=CARTESIAN_POINT('Ctrl Pts',(20.1804511070728,17.0971287527976,-6.29031796905216));
#49870=CARTESIAN_POINT('Ctrl Pts',(20.1095244508951,17.0519417597041,-6.29448768337254));
#49871=CARTESIAN_POINT('Ctrl Pts',(20.0386003185924,17.0067563745578,-6.29865724931658));
#49872=CARTESIAN_POINT('Ctrl Pts',(19.9654461005736,16.9650685803562,-6.30282681526061));
#49873=CARTESIAN_POINT('Ctrl Pts',(19.8904446404444,16.9270919909971,-6.30699638120464));
#49874=CARTESIAN_POINT('Ctrl Pts',(19.8128062215012,16.8877801916052,-6.31131254394357));
#49875=CARTESIAN_POINT('Ctrl Pts',(19.7331887160479,16.8524456628669,-6.31562870668249));
#49876=CARTESIAN_POINT('Ctrl Pts',(19.6520415805985,16.8212720539165,-6.31994486942141));
#49877=CARTESIAN_POINT('Ctrl Pts',(19.5735378045512,16.7911139219988,-6.32412043361309));
#49878=CARTESIAN_POINT('Ctrl Pts',(19.4936029857573,16.7648498911065,-6.32829599780477));
#49879=CARTESIAN_POINT('Ctrl Pts',(19.4126598398385,16.7425954906478,-6.33247156199645));
#49880=CARTESIAN_POINT('Ctrl Pts',(19.3276284480433,16.7192170733266,-6.33685802400899));
#49881=CARTESIAN_POINT('Ctrl Pts',(19.2414847611992,16.7002641097526,-6.34124448602154));
#49882=CARTESIAN_POINT('Ctrl Pts',(19.154729026295,16.6858094950216,-6.34563094803408));
#49883=CARTESIAN_POINT('Ctrl Pts',(19.0679732913908,16.6713548802907,-6.35001741004663));
#49884=CARTESIAN_POINT('Ctrl Pts',(18.9806060935248,16.6613986045227,-6.35440387205917));
#49885=CARTESIAN_POINT('Ctrl Pts',(18.8931294701917,16.6559505265619,-6.35879033407172));
#49886=CARTESIAN_POINT('Ctrl Pts',(18.8096777759695,16.650753122744,-6.36297496846477));
#49887=CARTESIAN_POINT('Ctrl Pts',(18.7258158815285,16.6496388297568,-6.36715960285782));
#49888=CARTESIAN_POINT('Ctrl Pts',(18.6419771668654,16.6526544802975,-6.37134423725087));
#49889=CARTESIAN_POINT('Ctrl Pts',(18.5582577862359,16.6556658384328,-6.3755229153348));
#49890=CARTESIAN_POINT('Ctrl Pts',(18.4745619756522,16.6627954472227,-6.37970159341873));
#49891=CARTESIAN_POINT('Ctrl Pts',(18.391326582379,16.6740382484444,-6.38388027150266));
#49892=CARTESIAN_POINT('Ctrl Pts',(18.3065992545013,16.6854825687981,-6.3881338493881));
#49893=CARTESIAN_POINT('Ctrl Pts',(18.2223494934534,16.7011890198916,-6.39238742727354));
#49894=CARTESIAN_POINT('Ctrl Pts',(18.1390363521675,16.7210967372691,-6.39664100515897));
#49895=CARTESIAN_POINT('Ctrl Pts',(18.0573383986977,16.7406185046986,-6.40081211913692));
#49896=CARTESIAN_POINT('Ctrl Pts',(17.9765415407101,16.7641799807696,-6.40498323311487));
#49897=CARTESIAN_POINT('Ctrl Pts',(17.8970700591987,16.7916719374606,-6.40915434709282));
#49898=CARTESIAN_POINT('Ctrl Pts',(17.8176252451106,16.81915466896,-6.41332406141319));
#49899=CARTESIAN_POINT('Ctrl Pts',(17.7395053586247,16.8505651114303,-6.41749377573355));
#49900=CARTESIAN_POINT('Ctrl Pts',(17.6631189946713,16.8857443425666,-6.42166349005392));
#49901=CARTESIAN_POINT('Ctrl Pts',(17.5867353488726,16.9209223218748,-6.42583305599795));
#49902=CARTESIAN_POINT('Ctrl Pts',(17.5120855204514,16.9598686299929,-6.43000262194199));
#49903=CARTESIAN_POINT('Ctrl Pts',(17.4395563508731,17.002376981186,-6.43417218788603));
#49904=CARTESIAN_POINT('Ctrl Pts',(17.3644771451667,17.0463798735675,-6.43848835062496));
#49905=CARTESIAN_POINT('Ctrl Pts',(17.2916709526717,17.0941996856766,-6.44280451336388));
#49906=CARTESIAN_POINT('Ctrl Pts',(17.2215354755333,17.1455579015064,-6.44712067610281));
#49907=CARTESIAN_POINT('Ctrl Pts',(17.1536846541857,17.1952431288574,-6.45129624029449));
#49908=CARTESIAN_POINT('Ctrl Pts',(17.0883335592488,17.2482394397185,-6.45547180448617));
#49909=CARTESIAN_POINT('Ctrl Pts',(17.0258081406205,17.3042539310255,-6.45964736867785));
#49910=CARTESIAN_POINT('Ctrl Pts',(16.9601247117373,17.3630975811266,-6.4640338306904));
#49911=CARTESIAN_POINT('Ctrl Pts',(16.8975603248985,17.4252719095173,-6.46842029270295));
#49912=CARTESIAN_POINT('Ctrl Pts',(16.8384470475511,17.4903957443787,-6.4728067547155));
#49913=CARTESIAN_POINT('Ctrl Pts',(16.7793337702037,17.55551957924,-6.47719321672805));
#49914=CARTESIAN_POINT('Ctrl Pts',(16.7236719107427,17.6235924232491,-6.4815796787406));
#49915=CARTESIAN_POINT('Ctrl Pts',(16.6717415022697,17.6941974787273,-6.48596614075315));
#49916=CARTESIAN_POINT('Ctrl Pts',(16.6219091295866,17.7619500256717,-6.4901753857061));
#49917=CARTESIAN_POINT('Ctrl Pts',(16.5753265021954,17.8322867639503,-6.49438463065906));
#49918=CARTESIAN_POINT('Ctrl Pts',(16.5322706261132,17.9048653345982,-6.49859387561201));
#49919=CARTESIAN_POINT('Ctrl Pts',(16.4892771418592,17.9773387323843,-6.50279702099131));
#49920=CARTESIAN_POINT('Ctrl Pts',(16.4498004872777,18.0520471246589,-6.5070001663706));
#49921=CARTESIAN_POINT('Ctrl Pts',(16.4140760664827,18.128617007389,-6.5112033117499));
#49922=CARTESIAN_POINT('Ctrl Pts',(16.3783931208862,18.2050979943158,-6.51540157737789));
#49923=CARTESIAN_POINT('Ctrl Pts',(16.3464539443372,18.2834357700826,-6.51959984300588));
#49924=CARTESIAN_POINT('Ctrl Pts',(16.3184487740251,18.3632310015746,-6.52379810863387));
#49925=CARTESIAN_POINT('Ctrl Pts',(16.2904693914728,18.4429527559108,-6.52799250840908));
#49926=CARTESIAN_POINT('Ctrl Pts',(16.2664169618498,18.5241288717768,-6.53218690818429));
#49927=CARTESIAN_POINT('Ctrl Pts',(16.2464336691667,18.6063399717985,-6.5363813079595));
#49928=CARTESIAN_POINT('Ctrl Pts',(16.2264610773219,18.6885070486605,-6.54057346167876));
#49929=CARTESIAN_POINT('Ctrl Pts',(16.210553397436,18.7717075687093,-6.54476561539801));
#49930=CARTESIAN_POINT('Ctrl Pts',(16.1988026788696,18.8555080269072,-6.54895776911726));
#49931=CARTESIAN_POINT('Ctrl Pts',(16.1870533030452,18.9392989093172,-6.55314944380363));
#49932=CARTESIAN_POINT('Ctrl Pts',(16.1794600117858,19.0236891460433,-6.55734111849001));
#49933=CARTESIAN_POINT('Ctrl Pts',(16.1760633700115,19.1082371810286,-6.56153279317638));
#49934=CARTESIAN_POINT('Ctrl Pts',(16.1746649834927,19.1430453357189,-6.56325849219375));
#49935=CARTESIAN_POINT('Ctrl Pts',(16.173977295445,19.1778801783156,-6.56498419121113));
#49936=CARTESIAN_POINT('Ctrl Pts',(16.1740005716256,19.2127107666517,-6.5667098902285));
#49937=CARTESIAN_POINT('Origin',(18.734,19.211,1.76670989022852));
#49938=CARTESIAN_POINT('',(20.2935358855687,21.2411349269503,-5.2501823431226));
#49939=CARTESIAN_POINT('',(20.2935358855687,21.2411349269503,-5.31661775129949));
#49940=CARTESIAN_POINT('',(20.2935358855687,21.2411349269503,1.76670989022852));
#49941=CARTESIAN_POINT('',(16.1740005630998,19.2126979607665,-5.83329010977151));
#49942=CARTESIAN_POINT('Ctrl Pts',(20.2935358855687,21.2411349269503,-5.31661775129949));
#49943=CARTESIAN_POINT('Ctrl Pts',(20.3601996618573,21.1899242660186,-5.32080132208221));
#49944=CARTESIAN_POINT('Ctrl Pts',(20.4242600608059,21.1354868005558,-5.32498489286492));
#49945=CARTESIAN_POINT('Ctrl Pts',(20.4854058680557,21.0781308163436,-5.32916846364764));
#49946=CARTESIAN_POINT('Ctrl Pts',(20.5380265760828,21.0287715448812,-5.33276875067579));
#49947=CARTESIAN_POINT('Ctrl Pts',(20.5884892422948,20.9772515834067,-5.33636903770395));
#49948=CARTESIAN_POINT('Ctrl Pts',(20.6366195645772,20.923786849695,-5.3399693247321));
#49949=CARTESIAN_POINT('Ctrl Pts',(20.6925617159657,20.8616444811129,-5.34415395912515));
#49950=CARTESIAN_POINT('Ctrl Pts',(20.7455602793472,20.7966428559979,-5.34833859351819));
#49951=CARTESIAN_POINT('Ctrl Pts',(20.7953091936645,20.7290923582293,-5.35252322791124));
#49952=CARTESIAN_POINT('Ctrl Pts',(20.8449872965599,20.6616380102333,-5.35670190599519));
#49953=CARTESIAN_POINT('Ctrl Pts',(20.891424667568,20.5916423631925,-5.36088058407913));
#49954=CARTESIAN_POINT('Ctrl Pts',(20.934353739878,20.5194507707228,-5.36505926216307));
#49955=CARTESIAN_POINT('Ctrl Pts',(20.9780522849565,20.4459651958412,-5.36931284004851));
#49956=CARTESIAN_POINT('Ctrl Pts',(21.0181151991572,20.3702045348863,-5.37356641793395));
#49957=CARTESIAN_POINT('Ctrl Pts',(21.0543048298795,20.2925662237874,-5.37781999581938));
#49958=CARTESIAN_POINT('Ctrl Pts',(21.089792853992,20.2164330828479,-5.38199110979733));
#49959=CARTESIAN_POINT('Ctrl Pts',(21.1215562334332,20.1384948820617,-5.38616222377529));
#49960=CARTESIAN_POINT('Ctrl Pts',(21.1494168148283,20.0591518794676,-5.39033333775324));
#49961=CARTESIAN_POINT('Ctrl Pts',(21.1772680473363,19.9798355011844,-5.39450305207361));
#49962=CARTESIAN_POINT('Ctrl Pts',(21.2012189304412,19.8991156909809,-5.39867276639398));
#49963=CARTESIAN_POINT('Ctrl Pts',(21.2211399893044,19.817411307285,-5.40284248071436));
#49964=CARTESIAN_POINT('Ctrl Pts',(21.2410603392908,19.7357098309816,-5.4070120466584));
#49965=CARTESIAN_POINT('Ctrl Pts',(21.2569510420042,19.6530242979867,-5.41118161260244));
#49966=CARTESIAN_POINT('Ctrl Pts',(21.2687332465284,19.5697859653662,-5.41535117854649));
#49967=CARTESIAN_POINT('Ctrl Pts',(21.2809296988287,19.4836210756563,-5.41966734128541));
#49968=CARTESIAN_POINT('Ctrl Pts',(21.2887232939913,19.396864312403,-5.42398350402433));
#49969=CARTESIAN_POINT('Ctrl Pts',(21.2920850129342,19.3100003363693,-5.42829966676325));
#49970=CARTESIAN_POINT('Ctrl Pts',(21.2953372242362,19.2259659452184,-5.43247523095493));
#49971=CARTESIAN_POINT('Ctrl Pts',(21.2944419142066,19.1418316894466,-5.43665079514661));
#49972=CARTESIAN_POINT('Ctrl Pts',(21.2894259327675,19.0580349643243,-5.44082635933829));
#49973=CARTESIAN_POINT('Ctrl Pts',(21.2841566060303,18.9700058658239,-5.44521282135083));
#49974=CARTESIAN_POINT('Ctrl Pts',(21.2743394628619,18.8823498716687,-5.44959928336338));
#49975=CARTESIAN_POINT('Ctrl Pts',(21.2600666971253,18.7955640342066,-5.45398574537592));
#49976=CARTESIAN_POINT('Ctrl Pts',(21.2457939313886,18.7087781967444,-5.45837220738846));
#49977=CARTESIAN_POINT('Ctrl Pts',(21.2270657409798,18.6228630666792,-5.462758669401));
#49978=CARTESIAN_POINT('Ctrl Pts',(21.2040345704695,18.5382970784324,-5.46714513141354));
#49979=CARTESIAN_POINT('Ctrl Pts',(21.1820630982548,18.4576220966617,-5.47132976580659));
#49980=CARTESIAN_POINT('Ctrl Pts',(21.1560941354244,18.377874545241,-5.47551440019964));
#49981=CARTESIAN_POINT('Ctrl Pts',(21.1262230006562,18.2994797779909,-5.47969903459269));
#49982=CARTESIAN_POINT('Ctrl Pts',(21.0963943837511,18.2211965959888,-5.48387771267663));
#49983=CARTESIAN_POINT('Ctrl Pts',(21.0626747898134,18.1442627996735,-5.48805639076058));
#49984=CARTESIAN_POINT('Ctrl Pts',(21.0252097777407,18.0690903037518,-5.49223506884452));
#49985=CARTESIAN_POINT('Ctrl Pts',(20.9870732322522,17.9925703948663,-5.49648864672996));
#49986=CARTESIAN_POINT('Ctrl Pts',(20.9450558013772,17.9178760152568,-5.50074222461539));
#49987=CARTESIAN_POINT('Ctrl Pts',(20.8993630289915,17.8454221176818,-5.50499580250083));
#49988=CARTESIAN_POINT('Ctrl Pts',(20.8545561001606,17.7743728802934,-5.50916691647878));
#49989=CARTESIAN_POINT('Ctrl Pts',(20.8062153221384,17.7054784349764,-5.51333803045673));
#49990=CARTESIAN_POINT('Ctrl Pts',(20.7545808175507,17.6391052326106,-5.51750914443469));
#49991=CARTESIAN_POINT('Ctrl Pts',(20.7029636394196,17.5727543024138,-5.52167885875506));
#49992=CARTESIAN_POINT('Ctrl Pts',(20.6480552119857,17.5089232977413,-5.52584857307543));
#49993=CARTESIAN_POINT('Ctrl Pts',(20.5901376466263,17.4479478065648,-5.53001828739581));
#49994=CARTESIAN_POINT('Ctrl Pts',(20.5322221422224,17.3869744851579,-5.53418785333985));
#49995=CARTESIAN_POINT('Ctrl Pts',(20.4712980302308,17.3288568081792,-5.53835741928389));
#49996=CARTESIAN_POINT('Ctrl Pts',(20.4076852490904,17.2738945080411,-5.54252698522793));
#49997=CARTESIAN_POINT('Ctrl Pts',(20.3418359210399,17.2169998012334,-5.54684314796685));
#49998=CARTESIAN_POINT('Ctrl Pts',(20.2731057379437,17.163486830588,-5.55115931070577));
#49999=CARTESIAN_POINT('Ctrl Pts',(20.2018865153253,17.1136423342391,-5.55547547344469));
#50000=CARTESIAN_POINT('Ctrl Pts',(20.1329872513929,17.065421517116,-5.55965103763637));
#50001=CARTESIAN_POINT('Ctrl Pts',(20.0617590424853,17.0206340542481,-5.56382660182806));
#50002=CARTESIAN_POINT('Ctrl Pts',(19.9885842021593,16.979494122864,-5.56800216601974));
#50003=CARTESIAN_POINT('Ctrl Pts',(19.9117134746051,16.9362763113467,-5.57238862803228));
#50004=CARTESIAN_POINT('Ctrl Pts',(19.8326948219823,16.8970844480459,-5.57677509004481));
#50005=CARTESIAN_POINT('Ctrl Pts',(19.7519960894444,16.8621100575217,-5.58116155205735));
#50006=CARTESIAN_POINT('Ctrl Pts',(19.6712973569065,16.8271356669974,-5.58554801406989));
#50007=CARTESIAN_POINT('Ctrl Pts',(19.5889191146258,16.7963788809358,-5.58993447608243));
#50008=CARTESIAN_POINT('Ctrl Pts',(19.5053461655915,16.7699704850561,-5.59432093809497));
#50009=CARTESIAN_POINT('Ctrl Pts',(19.4256185318271,16.7447771786174,-5.59850557248802));
#50010=CARTESIAN_POINT('Ctrl Pts',(19.3445069543662,16.7234471296282,-5.60269020688107));
#50011=CARTESIAN_POINT('Ctrl Pts',(19.2624206826507,16.7061304261206,-5.60687484127411));
#50012=CARTESIAN_POINT('Ctrl Pts',(19.1804512505827,16.688838370797,-5.61105351935806));
#50013=CARTESIAN_POINT('Ctrl Pts',(19.097510326263,16.6755484082766,-5.615232197442));
#50014=CARTESIAN_POINT('Ctrl Pts',(19.0140230530434,16.6663611081797,-5.61941087552595));
#50015=CARTESIAN_POINT('Ctrl Pts',(18.9290393304527,16.6570091323315,-5.62366445341138));
#50016=CARTESIAN_POINT('Ctrl Pts',(18.8434899394339,16.651908491303,-5.62791803129682));
#50017=CARTESIAN_POINT('Ctrl Pts',(18.7578350465908,16.6511109612809,-5.63217160918225));
#50018=CARTESIAN_POINT('Ctrl Pts',(18.6738407409872,16.6503288929346,-5.6363427231602));
#50019=CARTESIAN_POINT('Ctrl Pts',(18.58974546897,16.6536845805936,-5.64051383713816));
#50020=CARTESIAN_POINT('Ctrl Pts',(18.5059873315598,16.6611744720411,-5.64468495111611));
#50021=CARTESIAN_POINT('Ctrl Pts',(18.4222573000016,16.6686618501832,-5.64885466543648));
#50022=CARTESIAN_POINT('Ctrl Pts',(18.3388646361981,16.6802806360296,-5.65302437975685));
#50023=CARTESIAN_POINT('Ctrl Pts',(18.2562442180638,16.6959752659613,-5.65719409407723));
#50024=CARTESIAN_POINT('Ctrl Pts',(18.1736267399186,16.7116693374106,-5.66136366002127));
#50025=CARTESIAN_POINT('Ctrl Pts',(18.0917819045974,16.7314388778862,-5.66553322596531));
#50026=CARTESIAN_POINT('Ctrl Pts',(18.0111349162343,16.7551771092621,-5.66970279190935));
#50027=CARTESIAN_POINT('Ctrl Pts',(17.9276524792492,16.7797499475689,-5.67401895464827));
#50028=CARTESIAN_POINT('Ctrl Pts',(17.8454541950085,16.8085755987089,-5.67833511738719));
#50029=CARTESIAN_POINT('Ctrl Pts',(17.7649932472177,16.8414798137466,-5.68265128012612));
#50030=CARTESIAN_POINT('Ctrl Pts',(17.6871533063383,16.8733121774403,-5.6868268443178));
#50031=CARTESIAN_POINT('Ctrl Pts',(17.6109396593041,16.9089612248341,-5.69100240850948));
#50032=CARTESIAN_POINT('Ctrl Pts',(17.5367393343476,16.9482214208011,-5.69517797270115));
#50033=CARTESIAN_POINT('Ctrl Pts',(17.458791327372,16.989464555934,-5.6995644347137));
#50034=CARTESIAN_POINT('Ctrl Pts',(17.3830658746254,17.0346929255447,-5.70395089672624));
#50035=CARTESIAN_POINT('Ctrl Pts',(17.3099772536615,17.0836168145088,-5.70833735873878));
#50036=CARTESIAN_POINT('Ctrl Pts',(17.2368886326976,17.1325407034729,-5.71272382075132));
#50037=CARTESIAN_POINT('Ctrl Pts',(17.1664372628671,17.185159703645,-5.71711028276386));
#50038=CARTESIAN_POINT('Ctrl Pts',(17.0989955289255,17.2411369642621,-5.72149674477641));
#50039=CARTESIAN_POINT('Ctrl Pts',(17.0355419517776,17.2938040179914,-5.72562381401755));
#50040=CARTESIAN_POINT('Ctrl Pts',(16.9745020021859,17.3496514870446,-5.72975088325869));
#50041=CARTESIAN_POINT('Ctrl Pts',(16.9162185170908,17.4084267059583,-5.73387795249983));
#50042=CARTESIAN_POINT('Ctrl Pts',(16.8577217299028,17.4674170265802,-5.73802012571948));
#50043=CARTESIAN_POINT('Ctrl Pts',(16.8020020379166,17.5293563204315,-5.74216229893914));
#50044=CARTESIAN_POINT('Ctrl Pts',(16.7493744028763,17.5939467419898,-5.74630447215879));
#50045=CARTESIAN_POINT('Ctrl Pts',(16.6970742796338,17.658135205051,-5.75042086784546));
#50046=CARTESIAN_POINT('Ctrl Pts',(16.6478281605157,17.7249415391099,-5.75453726353214));
#50047=CARTESIAN_POINT('Ctrl Pts',(16.6019085746493,17.7940362905332,-5.75865365921882));
#50048=CARTESIAN_POINT('Ctrl Pts',(16.5560170315912,17.8630888462173,-5.76276754104799));
#50049=CARTESIAN_POINT('Ctrl Pts',(16.5134482524876,17.9344266527044,-5.76688142287718));
#50050=CARTESIAN_POINT('Ctrl Pts',(16.4744330306067,18.0076891046671,-5.77099530470636));
#50051=CARTESIAN_POINT('Ctrl Pts',(16.4354291736145,18.0809302157386,-5.77510798818765));
#50052=CARTESIAN_POINT('Ctrl Pts',(16.3999770407451,18.1560944409467,-5.77922067166894));
#50053=CARTESIAN_POINT('Ctrl Pts',(16.3682620211174,18.2327956168202,-5.78333335515023));
#50054=CARTESIAN_POINT('Ctrl Pts',(16.3361584999703,18.3104363640294,-5.78749641803534));
#50055=CARTESIAN_POINT('Ctrl Pts',(16.3078844956125,18.3896515290332,-5.79165948092045));
#50056=CARTESIAN_POINT('Ctrl Pts',(16.2835818660733,18.4700202641616,-5.79582254380555));
#50057=CARTESIAN_POINT('Ctrl Pts',(16.2595524301163,18.5494855487963,-5.79993880837771));
#50058=CARTESIAN_POINT('Ctrl Pts',(16.2394055983611,18.6300781193828,-5.80405507294986));
#50059=CARTESIAN_POINT('Ctrl Pts',(16.2232275631063,18.7113783730311,-5.80817133752201));
#50060=CARTESIAN_POINT('Ctrl Pts',(16.2067736327736,18.7940650953989,-5.81235779956359));
#50061=CARTESIAN_POINT('Ctrl Pts',(16.1944252132088,18.877483359597,-5.81654426160518));
#50062=CARTESIAN_POINT('Ctrl Pts',(16.186218055036,18.9611857471735,-5.82073072364676));
#50063=CARTESIAN_POINT('Ctrl Pts',(16.1780108968631,19.04488813475,-5.82491718568835));
#50064=CARTESIAN_POINT('Ctrl Pts',(16.1739449655996,19.1288741338656,-5.82910364772993));
#50065=CARTESIAN_POINT('Ctrl Pts',(16.1740005630998,19.2126979607665,-5.83329010977151));
#50066=CARTESIAN_POINT('Ctrl Pts',(16.1712326816491,19.2126997966084,-5.83329010977151));
#50067=CARTESIAN_POINT('Ctrl Pts',(16.1704460797826,19.3154768238875,-5.83841759033362));
#50068=CARTESIAN_POINT('Ctrl Pts',(16.2227680075723,20.2671650151133,-5.88593700645621));
#50069=CARTESIAN_POINT('Ctrl Pts',(17.4141948907083,21.935225591005,-5.97584835813926));
#50070=CARTESIAN_POINT('Ctrl Pts',(19.4492535151759,21.8369133510816,-6.06521460816749));
#50071=CARTESIAN_POINT('Ctrl Pts',(20.2230158477614,21.3000309188846,-6.11218892263521));
#50072=CARTESIAN_POINT('Ctrl Pts',(20.2954006757859,21.2435252751206,-6.11677130154247));
#50073=CARTESIAN_POINT('',(16.1740007055014,19.2090994299067,-5.76670989019962));
#50074=CARTESIAN_POINT('Ctrl Pts',(16.174000705501,19.2090994304895,-5.76670989022851));
#50075=CARTESIAN_POINT('Ctrl Pts',(16.1739381768052,19.293323351932,-5.77088500205647));
#50076=CARTESIAN_POINT('Ctrl Pts',(16.1780364138872,19.3775880720651,-5.77506011388443));
#50077=CARTESIAN_POINT('Ctrl Pts',(16.1862808495761,19.4614538491682,-5.77923522571239));
#50078=CARTESIAN_POINT('Ctrl Pts',(16.1945245019763,19.5453116583386,-5.78340994087067));
#50079=CARTESIAN_POINT('Ctrl Pts',(16.2069135252696,19.6287701442273,-5.78758465602896));
#50080=CARTESIAN_POINT('Ctrl Pts',(16.223381442754,19.7113943045357,-5.79175937118724));
#50081=CARTESIAN_POINT('Ctrl Pts',(16.2398526754153,19.7940350980167,-5.79593492676263));
#50082=CARTESIAN_POINT('Ctrl Pts',(16.2604043427346,19.8758407835677,-5.80011048233803));
#50083=CARTESIAN_POINT('Ctrl Pts',(16.2849190524509,19.9563874914111,-5.80428603791342));
#50084=CARTESIAN_POINT('Ctrl Pts',(16.3094630809744,20.0370305305357,-5.80846658731946));
#50085=CARTESIAN_POINT('Ctrl Pts',(16.3379794801115,20.1164111473512,-5.8126471367255));
#50086=CARTESIAN_POINT('Ctrl Pts',(16.3703013760236,20.1941219736187,-5.81682768613154));
#50087=CARTESIAN_POINT('Ctrl Pts',(16.4026440716426,20.2718828081661,-5.82101092579446));
#50088=CARTESIAN_POINT('Ctrl Pts',(16.4387969424261,20.3479712998167,-5.82519416545737));
#50089=CARTESIAN_POINT('Ctrl Pts',(16.4785465454201,20.4220035979401,-5.82937740512028));
#50090=CARTESIAN_POINT('Ctrl Pts',(16.5183679957904,20.4961697093842,-5.83356820598561));
#50091=CARTESIAN_POINT('Ctrl Pts',(16.5617989238518,20.5682718138333,-5.83775900685093));
#50092=CARTESIAN_POINT('Ctrl Pts',(16.6085819963923,20.6379542073733,-5.84194980771626));
#50093=CARTESIAN_POINT('Ctrl Pts',(16.6388616407129,20.6830550948785,-5.84466224092616));
#50094=CARTESIAN_POINT('Ctrl Pts',(16.6705446814796,20.7271429654286,-5.84737467413607));
#50095=CARTESIAN_POINT('Ctrl Pts',(16.7035527014987,20.770129169764,-5.85008710734598));
#50096=CARTESIAN_POINT('Ctrl Pts',(16.754476165831,20.8364465811684,-5.85427174173903));
#50097=CARTESIAN_POINT('Ctrl Pts',(16.8087468503131,20.900389929485,-5.85845637613208));
#50098=CARTESIAN_POINT('Ctrl Pts',(16.8661152556941,20.9616017771011,-5.86264101052512));
#50099=CARTESIAN_POINT('Ctrl Pts',(16.9234020042509,21.0227264972286,-5.86681968860907));
#50100=CARTESIAN_POINT('Ctrl Pts',(16.9837774037105,21.0811271065654,-5.87099836669302));
#50101=CARTESIAN_POINT('Ctrl Pts',(17.0469505633859,21.1364776546146,-5.87517704477697));
#50102=CARTESIAN_POINT('Ctrl Pts',(17.1112560565466,21.1928203214578,-5.8794306226624));
#50103=CARTESIAN_POINT('Ctrl Pts',(17.1784603025303,21.2460021244014,-5.88368420054784));
#50104=CARTESIAN_POINT('Ctrl Pts',(17.2482157539324,21.2957170489391,-5.88793777843327));
#50105=CARTESIAN_POINT('Ctrl Pts',(17.3166188597925,21.344468152654,-5.89210889241122));
#50106=CARTESIAN_POINT('Ctrl Pts',(17.3874747417498,21.389885323497,-5.89628000638917));
#50107=CARTESIAN_POINT('Ctrl Pts',(17.4604222489457,21.4317205389286,-5.90045112036712));
#50108=CARTESIAN_POINT('Ctrl Pts',(17.5333452779011,21.4735417161497,-5.9046208346875));
#50109=CARTESIAN_POINT('Ctrl Pts',(17.6083581394478,21.5117830963987,-5.90879054900787));
#50110=CARTESIAN_POINT('Ctrl Pts',(17.6850725337914,21.5462411375773,-5.91296026332824));
#50111=CARTESIAN_POINT('Ctrl Pts',(17.7617841983077,21.5806979525909,-5.91712982927229));
#50112=CARTESIAN_POINT('Ctrl Pts',(17.8401968552433,21.6113715084928,-5.92129939521633));
#50113=CARTESIAN_POINT('Ctrl Pts',(17.9199007999998,21.6381057852016,-5.92546896116037));
#50114=CARTESIAN_POINT('Ctrl Pts',(18.0024070371285,21.6657800060992,-5.92978512389929));
#50115=CARTESIAN_POINT('Ctrl Pts',(18.0862965548757,21.6892326159303,-5.93410128663821));
#50116=CARTESIAN_POINT('Ctrl Pts',(18.1710980677304,21.7083468751151,-5.93841744937713));
#50117=CARTESIAN_POINT('Ctrl Pts',(18.2531371802234,21.7268384893174,-5.94259301356881));
#50118=CARTESIAN_POINT('Ctrl Pts',(18.3360293116301,21.7412700216399,-5.94676857776049));
#50119=CARTESIAN_POINT('Ctrl Pts',(18.4193394847882,21.751588270493,-5.95094414195217));
#50120=CARTESIAN_POINT('Ctrl Pts',(18.5068574567412,21.7624276695664,-5.95533060396471));
#50121=CARTESIAN_POINT('Ctrl Pts',(18.5948362284717,21.7687272994046,-5.95971706597725));
#50122=CARTESIAN_POINT('Ctrl Pts',(18.6827702698548,21.7704873538952,-5.96410352798979));
#50123=CARTESIAN_POINT('Ctrl Pts',(18.7707043112379,21.7722474083857,-5.96848999000233));
#50124=CARTESIAN_POINT('Ctrl Pts',(18.8585930447507,21.7694679818952,-5.97287645201487));
#50125=CARTESIAN_POINT('Ctrl Pts',(18.945938282031,21.7622119011579,-5.97726291402741));
#50126=CARTESIAN_POINT('Ctrl Pts',(19.0292570355293,21.7552903148054,-5.98144716675294));
#50127=CARTESIAN_POINT('Ctrl Pts',(19.1123913980882,21.744269959261,-5.98563141947847));
#50128=CARTESIAN_POINT('Ctrl Pts',(19.1949058912311,21.7291671428697,-5.989815672204));
#50129=CARTESIAN_POINT('Ctrl Pts',(19.2773086561187,21.7140847763564,-5.99399425926718));
#50130=CARTESIAN_POINT('Ctrl Pts',(19.3590927697212,21.6949310074223,-5.99817284633035));
#50131=CARTESIAN_POINT('Ctrl Pts',(19.4398267332542,21.6717739885296,-6.00235143339353));
#50132=CARTESIAN_POINT('Ctrl Pts',(19.5204679325005,21.6486435773276,-6.00652521921036));
#50133=CARTESIAN_POINT('Ctrl Pts',(19.6000609401169,21.6215191846142,-6.01069900502718));
#50134=CARTESIAN_POINT('Ctrl Pts',(19.6781847982248,21.5905199235983,-6.01487279084401));
#50135=CARTESIAN_POINT('Ctrl Pts',(19.7562551368422,21.5595418989204,-6.01904371736924));
#50136=CARTESIAN_POINT('Ctrl Pts',(19.8328578987203,21.5246944476579,-6.02321464389447));
#50137=CARTESIAN_POINT('Ctrl Pts',(19.9075887387111,21.4861460331967,-6.02738557041971));
#50138=CARTESIAN_POINT('Ctrl Pts',(19.9823054028883,21.4476049310463,-6.03155570575516));
#50139=CARTESIAN_POINT('Ctrl Pts',(20.0551504373937,21.4053644619575,-6.03572584109061));
#50140=CARTESIAN_POINT('Ctrl Pts',(20.1257419130185,21.3596401391456,-6.03989597642606));
#50141=CARTESIAN_POINT('Ctrl Pts',(20.1832317936462,21.3224021321912,-6.04329214544667));
#50142=CARTESIAN_POINT('Ctrl Pts',(20.2392273245281,21.2828543953029,-6.04668831446728));
#50143=CARTESIAN_POINT('Ctrl Pts',(20.2935358855687,21.2411349269503,-6.05008448348788));
#50144=CARTESIAN_POINT('Ctrl Pts',(20.2935358855687,21.2411349269503,-5.2501823431226));
#50145=CARTESIAN_POINT('Ctrl Pts',(20.3601377596623,21.1899718188651,-5.2543537748487));
#50146=CARTESIAN_POINT('Ctrl Pts',(20.4242723999887,21.1354869667526,-5.25852520657481));
#50147=CARTESIAN_POINT('Ctrl Pts',(20.4855962900899,21.0779521784297,-5.26269663830092));
#50148=CARTESIAN_POINT('Ctrl Pts',(20.5468968447462,21.020439283693,-5.2668664826813));
#50149=CARTESIAN_POINT('Ctrl Pts',(20.6053884380554,20.9598790719395,-5.27103632706169));
#50150=CARTESIAN_POINT('Ctrl Pts',(20.6607620024634,20.8965824470678,-5.27520617144207));
#50151=CARTESIAN_POINT('Ctrl Pts',(20.7161311064392,20.833290920844,-5.27937567993459));
#50152=CARTESIAN_POINT('Ctrl Pts',(20.7683823782338,20.7672637661809,-5.2835451884271));
#50153=CARTESIAN_POINT('Ctrl Pts',(20.8172458070711,20.6988463991019,-5.28771469691962));
#50154=CARTESIAN_POINT('Ctrl Pts',(20.866119957485,20.630414019936,-5.29188512028253));
#50155=CARTESIAN_POINT('Ctrl Pts',(20.9116045226243,20.5595907619903,-5.29605554364545));
#50156=CARTESIAN_POINT('Ctrl Pts',(20.9534725319694,20.4867514177274,-5.30022596700836));
#50157=CARTESIAN_POINT('Ctrl Pts',(20.9953878196887,20.4138298215057,-5.30440109971475));
#50158=CARTESIAN_POINT('Ctrl Pts',(21.0336781736472,20.3388879958581,-5.30857623242114));
#50159=CARTESIAN_POINT('Ctrl Pts',(21.0681626406287,20.2623252432493,-5.31275136512752));
#50160=CARTESIAN_POINT('Ctrl Pts',(21.1026701956664,20.1857112303112,-5.31692929317068));
#50161=CARTESIAN_POINT('Ctrl Pts',(21.1333666251999,20.1074745584388,-5.32110722121383));
#50162=CARTESIAN_POINT('Ctrl Pts',(21.1601200329157,20.0280321816703,-5.32528514925698));
#50163=CARTESIAN_POINT('Ctrl Pts',(21.1869161592313,19.9484629550019,-5.32946974842172));
#50164=CARTESIAN_POINT('Ctrl Pts',(21.2097565773899,19.8676846237838,-5.33365434758646));
#50165=CARTESIAN_POINT('Ctrl Pts',(21.228560023284,19.7861263254567,-5.3378389467512));
#50166=CARTESIAN_POINT('Ctrl Pts',(21.2338697291507,19.7630959416884,-5.33902059137422));
#50167=CARTESIAN_POINT('Ctrl Pts',(21.2388578511548,19.7400034037589,-5.34020223599723));
#50168=CARTESIAN_POINT('Ctrl Pts',(21.2435233083642,19.7168584434175,-5.34138388062024));
#50169=CARTESIAN_POINT('Ctrl Pts',(21.2600453931921,19.6348937010711,-5.34556851501328));
#50170=CARTESIAN_POINT('Ctrl Pts',(21.2725783676241,19.5519661209787,-5.34975314940633));
#50171=CARTESIAN_POINT('Ctrl Pts',(21.2810167729394,19.4684986570167,-5.35393778379938));
#50172=CARTESIAN_POINT('Ctrl Pts',(21.2894431672291,19.3851499986585,-5.35811646188331));
#50173=CARTESIAN_POINT('Ctrl Pts',(21.2937865229904,19.3012634366148,-5.36229513996725));
#50174=CARTESIAN_POINT('Ctrl Pts',(21.293992315731,19.2172724316081,-5.36647381805119));
#50175=CARTESIAN_POINT('Ctrl Pts',(21.2942017971586,19.1317759481998,-5.37072739593663));
#50176=CARTESIAN_POINT('Ctrl Pts',(21.2901238296771,19.0461717133525,-5.37498097382206));
#50177=CARTESIAN_POINT('Ctrl Pts',(21.2817561480521,18.9609227917973,-5.3792345517075));
#50178=CARTESIAN_POINT('Ctrl Pts',(21.2735506902637,18.877326586936,-5.38340566568545));
#50179=CARTESIAN_POINT('Ctrl Pts',(21.2612204100085,18.7940725203437,-5.38757677966341));
#50180=CARTESIAN_POINT('Ctrl Pts',(21.2448156932503,18.7115958004501,-5.39174789364136));
#50181=CARTESIAN_POINT('Ctrl Pts',(21.2284164812532,18.6291467564165,-5.39591760796173));
#50182=CARTESIAN_POINT('Ctrl Pts',(21.2079456377352,18.547474991856,-5.4000873222821));
#50183=CARTESIAN_POINT('Ctrl Pts',(21.18350491705,18.4670069480513,-5.40425703660247));
#50184=CARTESIAN_POINT('Ctrl Pts',(21.1590650660706,18.3865417676451,-5.4084266025465));
#50185=CARTESIAN_POINT('Ctrl Pts',(21.1306557533069,18.3072806627598,-5.41259616849054));
#50186=CARTESIAN_POINT('Ctrl Pts',(21.0984286192899,18.2296349790813,-5.41676573443457));
#50187=CARTESIAN_POINT('Ctrl Pts',(21.0650684189972,18.1492593689506,-5.4210818971735));
#50188=CARTESIAN_POINT('Ctrl Pts',(21.0276171353227,18.0706153771464,-5.42539805991242));
#50189=CARTESIAN_POINT('Ctrl Pts',(20.9862964849995,17.9941349525692,-5.42971422265135));
#50190=CARTESIAN_POINT('Ctrl Pts',(20.9463218505145,17.9201458697782,-5.43388978684303));
#50191=CARTESIAN_POINT('Ctrl Pts',(20.9027263517809,17.8481819408659,-5.43806535103471));
#50192=CARTESIAN_POINT('Ctrl Pts',(20.8557557370749,17.7786059926858,-5.44224091522639));
#50193=CARTESIAN_POINT('Ctrl Pts',(20.8064127482821,17.7055159287641,-5.44662737723894));
#50194=CARTESIAN_POINT('Ctrl Pts',(20.7533450801513,17.6350618855125,-5.45101383925148));
#50195=CARTESIAN_POINT('Ctrl Pts',(20.6968850924156,17.5676247799201,-5.45540030126403));
#50196=CARTESIAN_POINT('Ctrl Pts',(20.6404251046799,17.5001876743278,-5.45978676327658));
#50197=CARTESIAN_POINT('Ctrl Pts',(20.5805732479926,17.4357678796897,-5.46417322528913));
#50198=CARTESIAN_POINT('Ctrl Pts',(20.5177042670235,17.3746996193972,-5.46855968730167));
#50199=CARTESIAN_POINT('Ctrl Pts',(20.4577279810631,17.3164412002857,-5.47274432169472));
#50200=CARTESIAN_POINT('Ctrl Pts',(20.3947828711329,17.2610158259165,-5.47692895608776));
#50201=CARTESIAN_POINT('Ctrl Pts',(20.3291674917036,17.208741107296,-5.48111359048081));
#50202=CARTESIAN_POINT('Ctrl Pts',(20.2636455076451,17.156540795267,-5.48529226856476));
#50203=CARTESIAN_POINT('Ctrl Pts',(20.1954611603976,17.1074825154228,-5.48947094664871));
#50204=CARTESIAN_POINT('Ctrl Pts',(20.1249494087588,17.0618467383005,-5.49364962473266));
#50205=CARTESIAN_POINT('Ctrl Pts',(20.0531737846479,17.0153929726713,-5.4979032026181));
#50206=CARTESIAN_POINT('Ctrl Pts',(19.9789868438522,16.9724859492608,-5.50215678050353));
#50207=CARTESIAN_POINT('Ctrl Pts',(19.9027767244007,16.9333782209289,-5.50641035838897));
#50208=CARTESIAN_POINT('Ctrl Pts',(19.8280440868266,16.8950286722232,-5.51058147236691));
#50209=CARTESIAN_POINT('Ctrl Pts',(19.7513664452244,16.8603326394005,-5.51475258634486));
#50210=CARTESIAN_POINT('Ctrl Pts',(19.6731370139767,16.8294833259079,-5.51892370032281));
#50211=CARTESIAN_POINT('Ctrl Pts',(19.5949338333702,16.7986443642003,-5.52309341464318));
#50212=CARTESIAN_POINT('Ctrl Pts',(19.5151803248757,16.7716497268886,-5.52726312896355));
#50213=CARTESIAN_POINT('Ctrl Pts',(19.434290135828,16.7486446792427,-5.53143284328392));
#50214=CARTESIAN_POINT('Ctrl Pts',(19.3534028252003,16.725640450215,-5.53560240922796));
#50215=CARTESIAN_POINT('Ctrl Pts',(19.2713793571596,16.7066256536093,-5.53977197517201));
#50216=CARTESIAN_POINT('Ctrl Pts',(19.1886476884741,16.6916954373547,-5.54394154111605));
#50217=CARTESIAN_POINT('Ctrl Pts',(19.1030072763782,16.6762402931151,-5.54825770385497));
#50218=CARTESIAN_POINT('Ctrl Pts',(19.0166084554192,16.6651623947289,-5.5525738665939));
#50219=CARTESIAN_POINT('Ctrl Pts',(18.9299344373275,16.6585091192584,-5.55689002933282));
#50220=CARTESIAN_POINT('Ctrl Pts',(18.8460838162587,16.6520725735365,-5.5610655935245));
#50221=CARTESIAN_POINT('Ctrl Pts',(18.7619761239716,16.6497767790178,-5.56524115771618));
#50222=CARTESIAN_POINT('Ctrl Pts',(18.6780494593125,16.6516114915869,-5.56941672190786));
#50223=CARTESIAN_POINT('Ctrl Pts',(18.5898838583381,16.6535388711264,-5.5738031839204));
#50224=CARTESIAN_POINT('Ctrl Pts',(18.5019186353064,16.6600249445383,-5.57818964593294));
#50225=CARTESIAN_POINT('Ctrl Pts',(18.4146539811437,16.670996433026,-5.58257610794548));
#50226=CARTESIAN_POINT('Ctrl Pts',(18.3273893269809,16.6819679215137,-5.58696256995803));
#50227=CARTESIAN_POINT('Ctrl Pts',(18.2408257994993,16.6974246482065,-5.59134903197057));
#50228=CARTESIAN_POINT('Ctrl Pts',(18.1554472698611,16.7172324209243,-5.59573549398311));
#50229=CARTESIAN_POINT('Ctrl Pts',(18.073997132933,16.7361288086573,-5.59992012837615));
#50230=CARTESIAN_POINT('Ctrl Pts',(17.9933221701874,16.7590549809083,-5.6041047627692));
#50231=CARTESIAN_POINT('Ctrl Pts',(17.9138510440902,16.7859318174286,-5.60828939716224));
#50232=CARTESIAN_POINT('Ctrl Pts',(17.8344930353039,16.812770398099,-5.6124680752462));
#50233=CARTESIAN_POINT('Ctrl Pts',(17.7563358916492,16.8435483273115,-5.61664675333017));
#50234=CARTESIAN_POINT('Ctrl Pts',(17.6797967513065,16.878135771108,-5.62082543141413));
#50235=CARTESIAN_POINT('Ctrl Pts',(17.6018857018813,16.9133431699767,-5.62507900929956));
#50236=CARTESIAN_POINT('Ctrl Pts',(17.5256517013906,16.9524978888719,-5.629332587185));
#50237=CARTESIAN_POINT('Ctrl Pts',(17.4515171985758,16.9954102672085,-5.63358616507043));
#50238=CARTESIAN_POINT('Ctrl Pts',(17.3788199377597,17.0374907053544,-5.63775727904838));
#50239=CARTESIAN_POINT('Ctrl Pts',(17.3081419118292,17.0831841629374,-5.64192839302633));
#50240=CARTESIAN_POINT('Ctrl Pts',(17.2398584137958,17.1322645862508,-5.64609950700428));
#50241=CARTESIAN_POINT('Ctrl Pts',(17.1715978289495,17.1813285401541,-5.65026922132465));
#50242=CARTESIAN_POINT('Ctrl Pts',(17.1057305494612,17.2337769343487,-5.65443893564503));
#50243=CARTESIAN_POINT('Ctrl Pts',(17.0426026198909,17.2893405862224,-5.6586086499654));
#50244=CARTESIAN_POINT('Ctrl Pts',(16.9794769366833,17.3449022609028,-5.66277821590943));
#50245=CARTESIAN_POINT('Ctrl Pts',(16.9190907543426,17.4035786682712,-5.66694778185347));
#50246=CARTESIAN_POINT('Ctrl Pts',(16.8617557221014,17.4650614661805,-5.67111734779751));
#50247=CARTESIAN_POINT('Ctrl Pts',(16.8024048608568,17.5287059234172,-5.67543351053642));
#50248=CARTESIAN_POINT('Ctrl Pts',(16.7463240583277,17.5953574026463,-5.67974967327534));
#50249=CARTESIAN_POINT('Ctrl Pts',(16.6938147044704,17.6646352435778,-5.68406583601426));
#50250=CARTESIAN_POINT('Ctrl Pts',(16.643015837292,17.7316563661277,-5.68824140020594));
#50251=CARTESIAN_POINT('Ctrl Pts',(16.5955595388127,17.8011349549805,-5.69241696439763));
#50252=CARTESIAN_POINT('Ctrl Pts',(16.5516743299489,17.8726970933918,-5.69659252858931));
#50253=CARTESIAN_POINT('Ctrl Pts',(16.5055725835126,17.9478736652914,-5.70097899060185));
#50254=CARTESIAN_POINT('Ctrl Pts',(16.4634124379741,18.0253492855824,-5.70536545261439));
#50255=CARTESIAN_POINT('Ctrl Pts',(16.4254030213233,18.1046637084299,-5.70975191462692));
#50256=CARTESIAN_POINT('Ctrl Pts',(16.3873936046726,18.1839781312775,-5.71413837663946));
#50257=CARTESIAN_POINT('Ctrl Pts',(16.3535350701226,18.265130791913,-5.718524838652));
#50258=CARTESIAN_POINT('Ctrl Pts',(16.3239764935691,18.3476421955815,-5.72291130066454));
#50259=CARTESIAN_POINT('Ctrl Pts',(16.2911969765864,18.4391447059584,-5.72777574688621));
#50260=CARTESIAN_POINT('Ctrl Pts',(16.2636032939179,18.5325974942141,-5.73264019310788));
#50261=CARTESIAN_POINT('Ctrl Pts',(16.2413973788042,18.6274486545232,-5.73750463932955));
#50262=CARTESIAN_POINT('Ctrl Pts',(16.2191773325015,18.7223601753114,-5.74237218114123));
#50263=CARTESIAN_POINT('Ctrl Pts',(16.2023520711405,18.818671733483,-5.74723972295291));
#50264=CARTESIAN_POINT('Ctrl Pts',(16.191076093449,18.9158085274076,-5.75210726476459));
#50265=CARTESIAN_POINT('Ctrl Pts',(16.1798001157575,19.0129453213322,-5.75697480657626));
#50266=CARTESIAN_POINT('Ctrl Pts',(16.1740736044194,19.1109072194811,-5.76184234838794));
#50267=CARTESIAN_POINT('Ctrl Pts',(16.1740007055014,19.2090994299067,-5.76670989019962));
#50268=CARTESIAN_POINT('Origin',(18.734,19.211,1.76670989022852));
#50269=CARTESIAN_POINT('',(20.2961058327006,21.2444858570038,-4.45010593307017));
#50270=CARTESIAN_POINT('',(20.2910030748979,21.2378274151617,-4.51667470337929));
#50271=CARTESIAN_POINT('',(20.2935358855687,21.2411349269503,1.76670989022852));
#50272=CARTESIAN_POINT('',(16.1741505041835,19.2121967451321,-5.03329016024809));
#50273=CARTESIAN_POINT('Ctrl Pts',(20.2910030748979,21.2378274151617,-4.51667470337929));
#50274=CARTESIAN_POINT('Ctrl Pts',(20.6127492989713,20.9913952836578,-4.53675463046736));
#50275=CARTESIAN_POINT('Ctrl Pts',(21.4403820747963,20.0000799362034,-4.59922649311591));
#50276=CARTESIAN_POINT('Ctrl Pts',(21.3050299007693,17.61315900461,-4.70409029132493));
#50277=CARTESIAN_POINT('Ctrl Pts',(18.7821183085442,16.1842897024026,-4.83126609800637));
#50278=CARTESIAN_POINT('Ctrl Pts',(16.5671405518731,17.3473640177625,-4.94099937082189));
#50279=CARTESIAN_POINT('Ctrl Pts',(16.1797898343239,18.7088775035926,-5.00834070807693));
#50280=CARTESIAN_POINT('Ctrl Pts',(16.1776748250889,19.2121940791439,-5.0332901097715));
#50281=CARTESIAN_POINT('Ctrl Pts',(16.1740002797795,19.2121968587701,-5.03329016239966));
#50282=CARTESIAN_POINT('Ctrl Pts',(16.1740435234787,19.3046921980315,-5.03786858507908));
#50283=CARTESIAN_POINT('Ctrl Pts',(16.1791038614083,19.3970207371689,-5.0424470077585));
#50284=CARTESIAN_POINT('Ctrl Pts',(16.1891023385012,19.4886614710357,-5.04702543043792));
#50285=CARTESIAN_POINT('Ctrl Pts',(16.199131888135,19.5805869993194,-5.05161808160682));
#50286=CARTESIAN_POINT('Ctrl Pts',(16.2141301908471,19.6718201549905,-5.05621073277571));
#50287=CARTESIAN_POINT('Ctrl Pts',(16.2339673694789,19.7618510200861,-5.0608033839446));
#50288=CARTESIAN_POINT('Ctrl Pts',(16.2538962421947,19.8522980379953,-5.06541726388547));
#50289=CARTESIAN_POINT('Ctrl Pts',(16.2787086950664,19.9415313458139,-5.07003114382633));
#50290=CARTESIAN_POINT('Ctrl Pts',(16.3082244096461,20.0290542679085,-5.07464502376719));
#50291=CARTESIAN_POINT('Ctrl Pts',(16.331622411587,20.0984363421765,-5.07830258630121));
#50292=CARTESIAN_POINT('Ctrl Pts',(16.3579750606107,20.1667439285256,-5.08196014883522));
#50293=CARTESIAN_POINT('Ctrl Pts',(16.3871718743355,20.233740313369,-5.08561771136923));
#50294=CARTESIAN_POINT('Ctrl Pts',(16.4205760854035,20.310391190454,-5.08980234576228));
#50295=CARTESIAN_POINT('Ctrl Pts',(16.457801705802,20.385546444256,-5.09398698015532));
#50296=CARTESIAN_POINT('Ctrl Pts',(16.4986929228154,20.4587989704629,-5.09817161454837));
#50297=CARTESIAN_POINT('Ctrl Pts',(16.5395259362427,20.5319472307656,-5.10235029263232));
#50298=CARTESIAN_POINT('Ctrl Pts',(16.5840139603303,20.6031977447539,-5.10652897071627));
#50299=CARTESIAN_POINT('Ctrl Pts',(16.6319534129312,20.6721639695094,-5.11070764880021));
#50300=CARTESIAN_POINT('Ctrl Pts',(16.6807521457666,20.7423663642785,-5.11496122668565));
#50301=CARTESIAN_POINT('Ctrl Pts',(16.7331270652481,20.8102013305708,-5.11921480457108));
#50302=CARTESIAN_POINT('Ctrl Pts',(16.7888147952353,20.8752879916542,-5.12346838245652));
#50303=CARTESIAN_POINT('Ctrl Pts',(16.843422909911,20.9391128208063,-5.12763949643447));
#50304=CARTESIAN_POINT('Ctrl Pts',(16.9012162179244,21.0002945906744,-5.13181061041243));
#50305=CARTESIAN_POINT('Ctrl Pts',(16.9619041398262,21.0585054160556,-5.13598172439038));
#50306=CARTESIAN_POINT('Ctrl Pts',(17.0225716973097,21.1166967082321,-5.14015143871075));
#50307=CARTESIAN_POINT('Ctrl Pts',(17.0861316079122,21.1719187176575,-5.14432115303112));
#50308=CARTESIAN_POINT('Ctrl Pts',(17.1522562065727,21.2238801683047,-5.14849086735149));
#50309=CARTESIAN_POINT('Ctrl Pts',(17.2183784522363,21.2758397699405,-5.15266043329554));
#50310=CARTESIAN_POINT('Ctrl Pts',(17.2870648422625,21.3245387599152,-5.15682999923959));
#50311=CARTESIAN_POINT('Ctrl Pts',(17.3579554657573,21.3697268098999,-5.16099956518364));
#50312=CARTESIAN_POINT('Ctrl Pts',(17.4313385161211,21.4165036159766,-5.16531572792256));
#50313=CARTESIAN_POINT('Ctrl Pts',(17.5070832408528,21.4595177156541,-5.16963189066148));
#50314=CARTESIAN_POINT('Ctrl Pts',(17.5847604857698,21.4985420299815,-5.1739480534004));
#50315=CARTESIAN_POINT('Ctrl Pts',(17.6599074026039,21.5362951313744,-5.17812361759208));
#50316=CARTESIAN_POINT('Ctrl Pts',(17.7368624194981,21.5703142429023,-5.18229918178376));
#50317=CARTESIAN_POINT('Ctrl Pts',(17.8152162748905,21.6004427104398,-5.18647474597544));
#50318=CARTESIAN_POINT('Ctrl Pts',(17.8975275972502,21.632092895249,-5.19086120798798));
#50319=CARTESIAN_POINT('Ctrl Pts',(17.9813822273946,21.6594488930309,-5.19524767000052));
#50320=CARTESIAN_POINT('Ctrl Pts',(18.0662895457781,21.6823888300554,-5.19963413201305));
#50321=CARTESIAN_POINT('Ctrl Pts',(18.1511968641616,21.70532876708,-5.20402059402559));
#50322=CARTESIAN_POINT('Ctrl Pts',(18.2371562875637,21.723852595477,-5.20840705603813));
#50323=CARTESIAN_POINT('Ctrl Pts',(18.3236691980734,21.7379009939035,-5.21279351805067));
#50324=CARTESIAN_POINT('Ctrl Pts',(18.408989825629,21.7517557834699,-5.21711952776937));
#50325=CARTESIAN_POINT('Ctrl Pts',(18.4951771222118,21.7613111070864,-5.22144553748807));
#50326=CARTESIAN_POINT('Ctrl Pts',(18.5817594759544,21.7664691981783,-5.22577154720677));
#50327=CARTESIAN_POINT('Ctrl Pts',(18.6653746425121,21.7714505208975,-5.22994930407667));
#50328=CARTESIAN_POINT('Ctrl Pts',(18.7493577223217,21.7723310236273,-5.23412706094656));
#50329=CARTESIAN_POINT('Ctrl Pts',(18.8332735539207,21.7690744245412,-5.23830481781645));
#50330=CARTESIAN_POINT('Ctrl Pts',(18.9171071868207,21.7658210154159,-5.24247848241707));
#50331=CARTESIAN_POINT('Ctrl Pts',(19.0008732452765,21.7584385686514,-5.24665214701768));
#50332=CARTESIAN_POINT('Ctrl Pts',(19.0841345036665,21.7469427890515,-5.2508258116183));
#50333=CARTESIAN_POINT('Ctrl Pts',(19.167339184286,21.7354548210748,-5.25499664012632));
#50334=CARTESIAN_POINT('Ctrl Pts',(19.2500392918514,21.7198591351502,-5.25916746863435));
#50335=CARTESIAN_POINT('Ctrl Pts',(19.3318020308339,21.7002233190156,-5.26333829714237));
#50336=CARTESIAN_POINT('Ctrl Pts',(19.4135337382729,21.6805949552937,-5.26750754268916));
#50337=CARTESIAN_POINT('Ctrl Pts',(19.4943283376287,21.6569296169492,-5.27167678823594));
#50338=CARTESIAN_POINT('Ctrl Pts',(19.5737638923663,21.6293458406683,-5.27584603378273));
#50339=CARTESIAN_POINT('Ctrl Pts',(19.6532187793364,21.6017553513233,-5.28001629399888));
#50340=CARTESIAN_POINT('Ctrl Pts',(19.7313135243688,21.5702446646857,-5.28418655421504));
#50341=CARTESIAN_POINT('Ctrl Pts',(19.8076429172256,21.5349816880284,-5.28835681443119));
#50342=CARTESIAN_POINT('Ctrl Pts',(19.8839842507333,21.4997131949786,-5.29252772702541));
#50343=CARTESIAN_POINT('Ctrl Pts',(19.9585592699248,21.4606914475138,-5.29669863961962));
#50344=CARTESIAN_POINT('Ctrl Pts',(20.0309859635671,21.4181310360533,-5.30086955221384));
#50345=CARTESIAN_POINT('Ctrl Pts',(20.1034742979777,21.3755344023614,-5.30504401458015));
#50346=CARTESIAN_POINT('Ctrl Pts',(20.1738102692344,21.3293933401784,-5.30921847694646));
#50347=CARTESIAN_POINT('Ctrl Pts',(20.2416402519882,21.2799661356787,-5.31339293931278));
#50348=CARTESIAN_POINT('Ctrl Pts',(20.2591066881619,21.2672384734032,-5.31446787664168));
#50349=CARTESIAN_POINT('Ctrl Pts',(20.2764071251532,21.25429312456,-5.31554281397059));
#50350=CARTESIAN_POINT('Ctrl Pts',(20.2935358855687,21.2411349269503,-5.31661775129949));
#50351=CARTESIAN_POINT('',(16.1737368487789,19.2101644346317,-4.96670989022851));
#50352=CARTESIAN_POINT('Ctrl Pts',(16.1740001363332,19.210164520558,-4.96670989022851));
#50353=CARTESIAN_POINT('Ctrl Pts',(16.1739730621524,19.2931227545131,-4.97085977152528));
#50354=CARTESIAN_POINT('Ctrl Pts',(16.1779827035226,19.3762448671897,-4.97500965282206));
#50355=CARTESIAN_POINT('Ctrl Pts',(16.1860506816107,19.4591013319584,-4.97915953411883));
#50356=CARTESIAN_POINT('Ctrl Pts',(16.194107496698,19.5418431550195,-4.98330367356457));
#50357=CARTESIAN_POINT('Ctrl Pts',(16.2062114544436,19.6243195978693,-4.9874478130103));
#50358=CARTESIAN_POINT('Ctrl Pts',(16.2223321624273,19.7061006702712,-4.99159195245604));
#50359=CARTESIAN_POINT('Ctrl Pts',(16.2384354396281,19.7877933155319,-4.99573161098225));
#50360=CARTESIAN_POINT('Ctrl Pts',(16.2585467481878,19.8687916269891,-4.99987126950846));
#50361=CARTESIAN_POINT('Ctrl Pts',(16.2825840079949,19.9486717658564,-5.00401092803467));
#50362=CARTESIAN_POINT('Ctrl Pts',(16.3066073287287,20.0285055826754,-5.00814818599591));
#50363=CARTESIAN_POINT('Ctrl Pts',(16.3345519481597,20.1072220663068,-5.01228544395717));
#50364=CARTESIAN_POINT('Ctrl Pts',(16.3662852025772,20.1844097996554,-5.01642270191841));
#50365=CARTESIAN_POINT('Ctrl Pts',(16.398009961529,20.2615768686959,-5.02055885227397));
#50366=CARTESIAN_POINT('Ctrl Pts',(16.4335211635115,20.3372155671951,-5.02469500262952));
#50367=CARTESIAN_POINT('Ctrl Pts',(16.4726375176033,20.4109332161453,-5.02883115298508));
#50368=CARTESIAN_POINT('Ctrl Pts',(16.5117556109319,20.4846541428151,-5.03296748724695));
#50369=CARTESIAN_POINT('Ctrl Pts',(16.5544789534247,20.5564534375443,-5.03710382150882));
#50370=CARTESIAN_POINT('Ctrl Pts',(16.6005803897988,20.6259631680044,-5.04124015577069));
#50371=CARTESIAN_POINT('Ctrl Pts',(16.6467285005472,20.6955432720456,-5.04538067777221));
#50372=CARTESIAN_POINT('Ctrl Pts',(16.6962612737686,20.7628287929976,-5.04952119977374));
#50373=CARTESIAN_POINT('Ctrl Pts',(16.7489086678718,20.827481488638,-5.05366172177526));
#50374=CARTESIAN_POINT('Ctrl Pts',(16.8015842228015,20.8921687666805,-5.0578044585212));
#50375=CARTESIAN_POINT('Ctrl Pts',(16.8573774008546,20.9542200685977,-5.06194719526713));
#50376=CARTESIAN_POINT('Ctrl Pts',(16.9159800655225,21.0133327988588,-5.06608993201307));
#50377=CARTESIAN_POINT('Ctrl Pts',(16.9746826938387,21.0725463628314,-5.07023973538442));
#50378=CARTESIAN_POINT('Ctrl Pts',(17.0362040315226,21.1288110311767,-5.07438953875576));
#50379=CARTESIAN_POINT('Ctrl Pts',(17.1002018437174,21.1818636646221,-5.07853934212711));
#50380=CARTESIAN_POINT('Ctrl Pts',(17.1438608301668,21.2180559050325,-5.08137031717053));
#50381=CARTESIAN_POINT('Ctrl Pts',(17.1886716656524,21.2527541562677,-5.08420129221395));
#50382=CARTESIAN_POINT('Ctrl Pts',(17.2345184376715,21.2858867545572,-5.08703226725736));
#50383=CARTESIAN_POINT('Ctrl Pts',(17.302287307428,21.3348620398235,-5.09121690165041));
#50384=CARTESIAN_POINT('Ctrl Pts',(17.3725842232475,21.38060482739,-5.09540153604346));
#50385=CARTESIAN_POINT('Ctrl Pts',(17.4450678487465,21.4228440065848,-5.09958617043651));
#50386=CARTESIAN_POINT('Ctrl Pts',(17.5174483027762,21.4650230635361,-5.10376484852045));
#50387=CARTESIAN_POINT('Ctrl Pts',(17.5920088899903,21.5037081881329,-5.10794352660439));
#50388=CARTESIAN_POINT('Ctrl Pts',(17.6683776217253,21.53867028312,-5.11212220468833));
#50389=CARTESIAN_POINT('Ctrl Pts',(17.7461152080914,21.574259048533,-5.11637578257376));
#50390=CARTESIAN_POINT('Ctrl Pts',(17.8257260077701,21.6059897185084,-5.1206293604592));
#50391=CARTESIAN_POINT('Ctrl Pts',(17.9067894477688,21.6336685085412,-5.12488293834464));
#50392=CARTESIAN_POINT('Ctrl Pts',(17.9862813148009,21.6608106912186,-5.12905405232259));
#50393=CARTESIAN_POINT('Ctrl Pts',(18.0671695448449,21.6840565436589,-5.13322516630054));
#50394=CARTESIAN_POINT('Ctrl Pts',(18.1490371223203,21.7032717411504,-5.1373962802785));
#50395=CARTESIAN_POINT('Ctrl Pts',(18.2308772283394,21.7224804907968,-5.14156599459887));
#50396=CARTESIAN_POINT('Ctrl Pts',(18.3136955816371,21.7376611666003,-5.14573570891925));
#50397=CARTESIAN_POINT('Ctrl Pts',(18.3970618790071,21.7487298324727,-5.14990542323963));
#50398=CARTESIAN_POINT('Ctrl Pts',(18.4804252098465,21.7597981044744,-5.15407498918367));
#50399=CARTESIAN_POINT('Ctrl Pts',(18.5643359898477,21.7667545977695,-5.15824455512772));
#50400=CARTESIAN_POINT('Ctrl Pts',(18.6483570024155,21.7695670358552,-5.16241412107176));
#50401=CARTESIAN_POINT('Ctrl Pts',(18.735332090134,21.7724783557944,-5.16673028381068));
#50402=CARTESIAN_POINT('Ctrl Pts',(18.8224247790693,21.7709487709587,-5.1710464465496));
#50403=CARTESIAN_POINT('Ctrl Pts',(18.9091500846463,21.7650012623036,-5.17536260928853));
#50404=CARTESIAN_POINT('Ctrl Pts',(18.993050322516,21.7592474931173,-5.1795381734802));
#50405=CARTESIAN_POINT('Ctrl Pts',(19.0766062822591,21.7493593099811,-5.18371373767188));
#50406=CARTESIAN_POINT('Ctrl Pts',(19.1593859487962,21.735410187463,-5.18788930186356));
#50407=CARTESIAN_POINT('Ctrl Pts',(19.2463466195001,21.7207565279273,-5.1922757638761));
#50408=CARTESIAN_POINT('Ctrl Pts',(19.3324499449363,21.7016210383821,-5.19666222588864));
#50409=CARTESIAN_POINT('Ctrl Pts',(19.4172115835234,21.6781485427796,-5.20104868790118));
#50410=CARTESIAN_POINT('Ctrl Pts',(19.5019732221104,21.6546760471771,-5.20543514991372));
#50411=CARTESIAN_POINT('Ctrl Pts',(19.5853926474676,21.6268668011754,-5.20982161192626));
#50412=CARTESIAN_POINT('Ctrl Pts',(19.6670104728636,21.5949235427183,-5.2142080739388));
#50413=CARTESIAN_POINT('Ctrl Pts',(19.7448664736172,21.5644525721622,-5.21839236074254));
#50414=CARTESIAN_POINT('Ctrl Pts',(19.821373063145,21.5301068697127,-5.22257664754627));
#50415=CARTESIAN_POINT('Ctrl Pts',(19.8961176236051,21.4920266611564,-5.22676093435));
#50416=CARTESIAN_POINT('Ctrl Pts',(19.9707478771509,21.4540046886926,-5.23093882212068));
#50417=CARTESIAN_POINT('Ctrl Pts',(20.0436210503422,21.4122597663648,-5.23511670989136));
#50418=CARTESIAN_POINT('Ctrl Pts',(20.1143433780777,21.3669805561732,-5.23929459766204));
#50419=CARTESIAN_POINT('Ctrl Pts',(20.1757784656169,21.3276474016958,-5.24292384614889));
#50420=CARTESIAN_POINT('Ctrl Pts',(20.2355906124235,21.2856480928829,-5.24655309463575));
#50421=CARTESIAN_POINT('Ctrl Pts',(20.2935358855687,21.2411349269503,-5.2501823431226));
#50422=CARTESIAN_POINT('Ctrl Pts',(20.296105832701,21.2444858570035,-4.4501059330702));
#50423=CARTESIAN_POINT('Ctrl Pts',(20.3016500430467,21.2402338391459,-4.4504550333302));
#50424=CARTESIAN_POINT('Ctrl Pts',(20.9781025843879,20.7166175212097,-4.49319606915068));
#50425=CARTESIAN_POINT('Ctrl Pts',(21.748497275926,18.9351410603846,-4.57832904053163));
#50426=CARTESIAN_POINT('Ctrl Pts',(20.1337364884029,16.526967633547,-4.70550484721307));
#50427=CARTESIAN_POINT('Ctrl Pts',(17.2348043502142,16.5812273130942,-4.8326806538945));
#50428=CARTESIAN_POINT('Ctrl Pts',(16.1917618195022,18.2701494080764,-4.91974900156632));
#50429=CARTESIAN_POINT('Ctrl Pts',(16.169904976237,19.1644257529645,-4.96442541367765));
#50430=CARTESIAN_POINT('Ctrl Pts',(16.170099683962,19.2101632476096,-4.96670989022851));
#50431=CARTESIAN_POINT('Origin',(18.734,19.211,1.76670989022852));
#50432=CARTESIAN_POINT('',(20.2935358855687,21.2411349269503,-3.65004596059139));
#50433=CARTESIAN_POINT('',(20.2935358855687,21.2411349269503,-3.71676815338605));
#50434=CARTESIAN_POINT('',(20.2935358855687,21.2411349269503,1.76670989022852));
#50435=CARTESIAN_POINT('',(16.1740009581142,19.2087851537238,-4.23329008724976));
#50436=CARTESIAN_POINT('Ctrl Pts',(20.2935358855687,21.2411349269503,-3.71676815338605));
#50437=CARTESIAN_POINT('Ctrl Pts',(20.3601013017359,21.1899998255969,-3.72094076519367));
#50438=CARTESIAN_POINT('Ctrl Pts',(20.4242136531026,21.1355378040453,-3.72511337700128));
#50439=CARTESIAN_POINT('Ctrl Pts',(20.4855270181563,21.0780171677487,-3.7292859888089));
#50440=CARTESIAN_POINT('Ctrl Pts',(20.5468083990537,21.020526537129,-3.73345642397089));
#50441=CARTESIAN_POINT('Ctrl Pts',(20.6052933577953,20.9599807738333,-3.73762685913287));
#50442=CARTESIAN_POINT('Ctrl Pts',(20.6606699248329,20.8966876937156,-3.74179729429485));
#50443=CARTESIAN_POINT('Ctrl Pts',(20.7160342164331,20.8334086439051,-3.74596680498789));
#50444=CARTESIAN_POINT('Ctrl Pts',(20.76829118238,20.7673838332093,-3.75013631568094));
#50445=CARTESIAN_POINT('Ctrl Pts',(20.817167476553,20.6989560694563,-3.75430582637399));
#50446=CARTESIAN_POINT('Ctrl Pts',(20.8660475978043,20.6305229477191,-3.75847566354522));
#50447=CARTESIAN_POINT('Ctrl Pts',(20.911546255344,20.5596868744331,-3.76264550071646));
#50448=CARTESIAN_POINT('Ctrl Pts',(20.9534327818709,20.4868205699693,-3.76681533788769));
#50449=CARTESIAN_POINT('Ctrl Pts',(20.9953632065693,20.4138778997194,-3.77098954515696));
#50450=CARTESIAN_POINT('Ctrl Pts',(21.0336737113649,20.3389011492554,-3.77516375242623));
#50451=CARTESIAN_POINT('Ctrl Pts',(21.0681793245512,20.2622882006557,-3.7793379596955));
#50452=CARTESIAN_POINT('Ctrl Pts',(21.1027036734523,20.1856336530745,-3.78351443345854));
#50453=CARTESIAN_POINT('Ctrl Pts',(21.133418848782,20.1073415667467,-3.78769090722157));
#50454=CARTESIAN_POINT('Ctrl Pts',(21.160188745424,20.0278281162997,-3.79186738098461));
#50455=CARTESIAN_POINT('Ctrl Pts',(21.1870051409859,19.9481765521498,-3.79605110922162));
#50456=CARTESIAN_POINT('Ctrl Pts',(21.2098624449983,19.867299829612,-3.80023483745864));
#50457=CARTESIAN_POINT('Ctrl Pts',(21.2286750191276,19.7856273130829,-3.80441856569565));
#50458=CARTESIAN_POINT('Ctrl Pts',(21.2428259538791,19.7241927404161,-3.80756559198206));
#50459=CARTESIAN_POINT('Ctrl Pts',(21.2546893788146,19.6623081668811,-3.81071261826848));
#50460=CARTESIAN_POINT('Ctrl Pts',(21.2642482087236,19.6001580684646,-3.81385964455489));
#50461=CARTESIAN_POINT('Ctrl Pts',(21.2769586867287,19.517516420223,-3.818044278948));
#50462=CARTESIAN_POINT('Ctrl Pts',(21.285639763102,19.4340976099862,-3.82222891334111));
#50463=CARTESIAN_POINT('Ctrl Pts',(21.2902056694013,19.350329019665,-3.82641354773422));
#50464=CARTESIAN_POINT('Ctrl Pts',(21.2947650766981,19.2666796635636,-3.83059222581822));
#50465=CARTESIAN_POINT('Ctrl Pts',(21.2952209238071,19.1826819717237,-3.83477090390223));
#50466=CARTESIAN_POINT('Ctrl Pts',(21.2915388082527,19.0987714640506,-3.83894958198623));
#50467=CARTESIAN_POINT('Ctrl Pts',(21.2877906934233,19.0133569208345,-3.84320315987165));
#50468=CARTESIAN_POINT('Ctrl Pts',(21.2797547375529,18.9280331946162,-3.84745673775707));
#50469=CARTESIAN_POINT('Ctrl Pts',(21.2674501116906,18.8432629586579,-3.85171031564249));
#50470=CARTESIAN_POINT('Ctrl Pts',(21.2553840350109,18.7601361591377,-3.85588142962051));
#50471=CARTESIAN_POINT('Ctrl Pts',(21.2392133934507,18.6775420566421,-3.86005254359852));
#50472=CARTESIAN_POINT('Ctrl Pts',(21.2190086634415,18.5959130609251,-3.86422365757653));
#50473=CARTESIAN_POINT('Ctrl Pts',(21.1988107133246,18.514311456606,-3.86839337189697));
#50474=CARTESIAN_POINT('Ctrl Pts',(21.1745814736228,18.4336747620778,-3.8725630862174));
#50475=CARTESIAN_POINT('Ctrl Pts',(21.1464423282956,18.3544242516579,-3.87673280053783));
#50476=CARTESIAN_POINT('Ctrl Pts',(21.1183041842799,18.2751765613113,-3.88090236648194));
#50477=CARTESIAN_POINT('Ctrl Pts',(21.0862565659976,18.197315390231,-3.88507193242604));
#50478=CARTESIAN_POINT('Ctrl Pts',(21.0504699913874,18.1212446242381,-3.88924149837015));
#50479=CARTESIAN_POINT('Ctrl Pts',(21.0134252049625,18.0424993039588,-3.893557661109));
#50480=CARTESIAN_POINT('Ctrl Pts',(20.9723738713788,17.965673109816,-3.89787382384785));
#50481=CARTESIAN_POINT('Ctrl Pts',(20.9275574633285,17.8911872651486,-3.9021899865867));
#50482=CARTESIAN_POINT('Ctrl Pts',(20.8842009450552,17.8191277890344,-3.90636555077843));
#50483=CARTESIAN_POINT('Ctrl Pts',(20.8373211816343,17.7492588949819,-3.91054111497017));
#50484=CARTESIAN_POINT('Ctrl Pts',(20.7871804520949,17.6819316460225,-3.91471667916191));
#50485=CARTESIAN_POINT('Ctrl Pts',(20.734507233507,17.6112038577767,-3.91910314117432));
#50486=CARTESIAN_POINT('Ctrl Pts',(20.6782353411158,17.5432816689316,-3.92348960318672));
#50487=CARTESIAN_POINT('Ctrl Pts',(20.6187144099126,17.4785302042842,-3.92787606519912));
#50488=CARTESIAN_POINT('Ctrl Pts',(20.5591934787095,17.4137787396368,-3.93226252721153));
#50489=CARTESIAN_POINT('Ctrl Pts',(20.4964239761435,17.3521983512227,-3.93664898922393));
#50490=CARTESIAN_POINT('Ctrl Pts',(20.4307957154099,17.2941055584183,-3.94103545123633));
#50491=CARTESIAN_POINT('Ctrl Pts',(20.3681871082353,17.2386857011236,-3.94522008562936));
#50492=CARTESIAN_POINT('Ctrl Pts',(20.3027439921319,17.1862332698865,-3.94940472002238));
#50493=CARTESIAN_POINT('Ctrl Pts',(20.2347793028206,17.137051716116,-3.95358935441541));
#50494=CARTESIAN_POINT('Ctrl Pts',(20.1669113528323,17.0879401661999,-3.95776803249933));
#50495=CARTESIAN_POINT('Ctrl Pts',(20.0965293283138,17.0420905134705,-3.96194671058325));
#50496=CARTESIAN_POINT('Ctrl Pts',(20.0239808111754,16.9997674236301,-3.96612538866717));
#50497=CARTESIAN_POINT('Ctrl Pts',(19.9501319140064,16.9566857228211,-3.97037896655261));
#50498=CARTESIAN_POINT('Ctrl Pts',(19.8740384525303,16.9172585752805,-3.97463254443805));
#50499=CARTESIAN_POINT('Ctrl Pts',(19.7960998386662,16.8817202974513,-3.9788861223235));
#50500=CARTESIAN_POINT('Ctrl Pts',(19.7196722169169,16.8468709984853,-3.98305723630143));
#50501=CARTESIAN_POINT('Ctrl Pts',(19.6414707859437,16.8157613278183,-3.98722835027936));
#50502=CARTESIAN_POINT('Ctrl Pts',(19.561897281475,16.7885660811229,-3.9913994642573));
#50503=CARTESIAN_POINT('Ctrl Pts',(19.4823504786642,16.7613799600552,-3.99556917857765));
#50504=CARTESIAN_POINT('Ctrl Pts',(19.4014329516943,16.7381058029317,-3.99973889289801));
#50505=CARTESIAN_POINT('Ctrl Pts',(19.3195646284335,16.7188695728499,-4.00390860721836));
#50506=CARTESIAN_POINT('Ctrl Pts',(19.2376992183989,16.6996340272756,-4.00807817316238));
#50507=CARTESIAN_POINT('Ctrl Pts',(19.1548835273743,16.6844362274532,-4.01224773910641));
#50508=CARTESIAN_POINT('Ctrl Pts',(19.0715494575451,16.6733514105158,-4.01641730505043));
#50509=CARTESIAN_POINT('Ctrl Pts',(18.9852854646236,16.6618768650894,-4.02073346778937));
#50510=CARTESIAN_POINT('Ctrl Pts',(18.8984664850875,16.6548099783526,-4.02504963052832));
#50511=CARTESIAN_POINT('Ctrl Pts',(18.8115774056933,16.6521757101892,-4.02936579326726));
#50512=CARTESIAN_POINT('Ctrl Pts',(18.7275187289222,16.6496272530341,-4.03354135745892));
#50513=CARTESIAN_POINT('Ctrl Pts',(18.643394919223,16.6512270080047,-4.03771692165058));
#50514=CARTESIAN_POINT('Ctrl Pts',(18.559643131712,16.6569444637047,-4.04189248584225));
#50515=CARTESIAN_POINT('Ctrl Pts',(18.4716612405136,16.6629506945001,-4.04627894785483));
#50516=CARTESIAN_POINT('Ctrl Pts',(18.3840905205399,16.6735014582054,-4.05066540986742));
#50517=CARTESIAN_POINT('Ctrl Pts',(18.2974272347526,16.6885004022509,-4.05505187188));
#50518=CARTESIAN_POINT('Ctrl Pts',(18.2107639489653,16.7034993462965,-4.05943833389259));
#50519=CARTESIAN_POINT('Ctrl Pts',(18.125008646392,16.7229462681819,-4.06382479590517));
#50520=CARTESIAN_POINT('Ctrl Pts',(18.040638468227,16.7466847226344,-4.06821125791776));
#50521=CARTESIAN_POINT('Ctrl Pts',(17.960150287027,16.7693309356085,-4.07239589231081));
#50522=CARTESIAN_POINT('Ctrl Pts',(17.8806229756134,16.7959667334644,-4.07658052670385));
#50523=CARTESIAN_POINT('Ctrl Pts',(17.8024810747699,16.8264932392761,-4.08076516109689));
#50524=CARTESIAN_POINT('Ctrl Pts',(17.7244503992502,16.8569762943851,-4.08494383918083));
#50525=CARTESIAN_POINT('Ctrl Pts',(17.6478016421982,16.8913388913935,-4.08912251726477));
#50526=CARTESIAN_POINT('Ctrl Pts',(17.5729454850808,16.9294320274457,-4.0933011953487));
#50527=CARTESIAN_POINT('Ctrl Pts',(17.496747585145,16.9682079555846,-4.09755477323414));
#50528=CARTESIAN_POINT('Ctrl Pts',(17.4224076460745,17.0108493474659,-4.10180835111958));
#50529=CARTESIAN_POINT('Ctrl Pts',(17.3503388850128,17.0571471919204,-4.10606192900502));
#50530=CARTESIAN_POINT('Ctrl Pts',(17.279667317515,17.1025474623173,-4.11023304298296));
#50531=CARTESIAN_POINT('Ctrl Pts',(17.2111800563177,17.1514634154306,-4.1144041569609));
#50532=CARTESIAN_POINT('Ctrl Pts',(17.1452415288499,17.2036518686713,-4.11857527093885));
#50533=CARTESIAN_POINT('Ctrl Pts',(17.0793251276917,17.2558228095726,-4.12274498525921));
#50534=CARTESIAN_POINT('Ctrl Pts',(17.0159561221395,17.3112637844565,-4.12691469957958));
#50535=CARTESIAN_POINT('Ctrl Pts',(16.9554677262144,17.3696898818767,-4.13108441389994));
#50536=CARTESIAN_POINT('Ctrl Pts',(16.8949814827259,17.4281139002458,-4.13525397984399));
#50537=CARTESIAN_POINT('Ctrl Pts',(16.8373759753513,17.4895225097358,-4.13942354578803));
#50538=CARTESIAN_POINT('Ctrl Pts',(16.7829482470742,17.5535932733921,-4.14359311173208));
#50539=CARTESIAN_POINT('Ctrl Pts',(16.7266069070147,17.6199166860587,-4.147909274471));
#50540=CARTESIAN_POINT('Ctrl Pts',(16.6736713066578,17.6890925366905,-4.15222543720993));
#50541=CARTESIAN_POINT('Ctrl Pts',(16.6244248933202,17.7607266225718,-4.15654159994886));
#50542=CARTESIAN_POINT('Ctrl Pts',(16.5767826767175,17.8300272356399,-4.16071716414053));
#50543=CARTESIAN_POINT('Ctrl Pts',(16.5325931948251,17.9016279637396,-4.16489272833221));
#50544=CARTESIAN_POINT('Ctrl Pts',(16.4920674161604,17.9751447133591,-4.16906829252389));
#50545=CARTESIAN_POINT('Ctrl Pts',(16.449494776756,18.0523746192327,-4.17345475453644));
#50546=CARTESIAN_POINT('Ctrl Pts',(16.4109659295263,18.1317186646457,-4.17784121654899));
#50547=CARTESIAN_POINT('Ctrl Pts',(16.3766684749371,18.2127074171643,-4.18222767856154));
#50548=CARTESIAN_POINT('Ctrl Pts',(16.342371020348,18.293696169683,-4.18661414057409));
#50549=CARTESIAN_POINT('Ctrl Pts',(16.3123050853067,18.3763290580522,-4.19100060258664));
#50550=CARTESIAN_POINT('Ctrl Pts',(16.2865973915759,18.4601202011779,-4.1953870645992));
#50551=CARTESIAN_POINT('Ctrl Pts',(16.256634152739,18.557781782967,-4.20049964335899));
#50552=CARTESIAN_POINT('Ctrl Pts',(16.2324986213398,18.6573099274652,-4.20561222211878));
#50553=CARTESIAN_POINT('Ctrl Pts',(16.2143850329176,18.7580757042789,-4.21072480087858));
#50554=CARTESIAN_POINT('Ctrl Pts',(16.1965183144929,18.8574681448718,-4.21576770033044));
#50555=CARTESIAN_POINT('Ctrl Pts',(16.184510545625,18.9580647258724,-4.2208105997823));
#50556=CARTESIAN_POINT('Ctrl Pts',(16.1785021632639,19.0592409592912,-4.22585349923416));
#50557=CARTESIAN_POINT('Ctrl Pts',(16.1755487125961,19.1089746473601,-4.22833236190603));
#50558=CARTESIAN_POINT('Ctrl Pts',(16.1740441624119,19.1588480714529,-4.23081122457789));
#50559=CARTESIAN_POINT('Ctrl Pts',(16.1740009581142,19.2087851537238,-4.23329008724976));
#50560=CARTESIAN_POINT('Ctrl Pts',(16.1756127741342,19.2087870016449,-4.2332901097715));
#50561=CARTESIAN_POINT('Ctrl Pts',(16.1805387735992,19.8078855990186,-4.26304769694121));
#50562=CARTESIAN_POINT('Ctrl Pts',(16.6895187210545,21.2679843244803,-4.3351972196714));
#50563=CARTESIAN_POINT('Ctrl Pts',(18.6971963258685,22.0472231898468,-4.429658750874));
#50564=CARTESIAN_POINT('Ctrl Pts',(19.9334915936059,21.5116529017718,-4.49436269490689));
#50565=CARTESIAN_POINT('Ctrl Pts',(20.2910030748979,21.2378274151617,-4.51667470337929));
#50566=CARTESIAN_POINT('',(16.1740010840393,19.2133559031925,-4.16670989022851));
#50567=CARTESIAN_POINT('Ctrl Pts',(16.1740881651155,19.2133565881468,-4.16670992828903));
#50568=CARTESIAN_POINT('Ctrl Pts',(16.1722334682522,19.4149927583358,-4.17674049235513));
#50569=CARTESIAN_POINT('Ctrl Pts',(16.2862272813843,20.4667260563269,-4.22916299198171));
#50570=CARTESIAN_POINT('Ctrl Pts',(17.7316712378677,22.0633000666069,-4.32362832690876));
#50571=CARTESIAN_POINT('Ctrl Pts',(19.628405606888,21.7565647837825,-4.40806309776972));
#50572=CARTESIAN_POINT('Ctrl Pts',(20.296105832701,21.2444858570035,-4.4501059330702));
#50573=CARTESIAN_POINT('Ctrl Pts',(20.2935358855687,21.2411349269503,-3.65004596059139));
#50574=CARTESIAN_POINT('Ctrl Pts',(20.3602232230616,21.1899061664612,-3.65422168157886));
#50575=CARTESIAN_POINT('Ctrl Pts',(20.4243341316756,21.1354261893531,-3.65839740256633));
#50576=CARTESIAN_POINT('Ctrl Pts',(20.4855499160717,21.077995685991,-3.6625731235538));
#50577=CARTESIAN_POINT('Ctrl Pts',(20.5479163689702,21.01948566577,-3.6668273352551));
#50578=CARTESIAN_POINT('Ctrl Pts',(20.6072773982079,20.9579134254356,-3.6710815469564));
#50579=CARTESIAN_POINT('Ctrl Pts',(20.6633380126266,20.8936333031989,-3.6753357586577));
#50580=CARTESIAN_POINT('Ctrl Pts',(20.7193986270453,20.8293531809622,-3.679589970359));
#50581=CARTESIAN_POINT('Ctrl Pts',(20.7721585712015,20.7623656090433,-3.6838441820603));
#50582=CARTESIAN_POINT('Ctrl Pts',(20.8213695361432,20.6930554711554,-3.6880983937616));
#50583=CARTESIAN_POINT('Ctrl Pts',(20.8697756595073,20.6248788952852,-3.69228302815506));
#50584=CARTESIAN_POINT('Ctrl Pts',(20.914928230553,20.5542014284548,-3.69646766254852));
#50585=CARTESIAN_POINT('Ctrl Pts',(20.956559006204,20.4813666651568,-3.70065229694198));
#50586=CARTESIAN_POINT('Ctrl Pts',(20.9981305255987,20.4086355731292,-3.70483097502633));
#50587=CARTESIAN_POINT('Ctrl Pts',(21.0361899803432,20.3337536798788,-3.70900965311069));
#50588=CARTESIAN_POINT('Ctrl Pts',(21.0705113959642,20.2570948793151,-3.71318833119504));
#50589=CARTESIAN_POINT('Ctrl Pts',(21.1054479982896,20.1790620248547,-3.71744190908037));
#50590=CARTESIAN_POINT('Ctrl Pts',(21.1365109555625,20.0991883275092,-3.72169548696571));
#50591=CARTESIAN_POINT('Ctrl Pts',(21.1635100116304,20.017895968132,-3.72594906485104));
#50592=CARTESIAN_POINT('Ctrl Pts',(21.1899856383154,19.9381796197602,-3.73012017882942));
#50593=CARTESIAN_POINT('Ctrl Pts',(21.2125533792702,19.8570995822363,-3.7342912928078));
#50594=CARTESIAN_POINT('Ctrl Pts',(21.2310824062636,19.7750739812551,-3.73846240678618));
#50595=CARTESIAN_POINT('Ctrl Pts',(21.249605215663,19.6930759047563,-3.74263212110698));
#50596=CARTESIAN_POINT('Ctrl Pts',(21.2640919013283,19.6101333433023,-3.74680183542779));
#50597=CARTESIAN_POINT('Ctrl Pts',(21.2744621331457,19.5266772878315,-3.7509715497486));
#50598=CARTESIAN_POINT('Ctrl Pts',(21.2848319959458,19.4432242020852,-3.75514111569308));
#50599=CARTESIAN_POINT('Ctrl Pts',(21.2910856402585,19.3592581152793,-3.75931068163755));
#50600=CARTESIAN_POINT('Ctrl Pts',(21.293194451632,19.2752164989407,-3.76348024758203));
#50601=CARTESIAN_POINT('Ctrl Pts',(21.2953774062114,19.1882200830675,-3.76779641032045));
#50602=CARTESIAN_POINT('Ctrl Pts',(21.2931186269949,19.1011432548625,-3.77211257305887));
#50603=CARTESIAN_POINT('Ctrl Pts',(21.2864451550249,19.0144707894738,-3.77642873579728));
#50604=CARTESIAN_POINT('Ctrl Pts',(21.2799890707009,18.9306216705101,-3.7806042999894));
#50605=CARTESIAN_POINT('Ctrl Pts',(21.2694016000863,18.847151436045,-3.78477986418152));
#50606=CARTESIAN_POINT('Ctrl Pts',(21.2547598325397,18.7644914707929,-3.78895542837365));
#50607=CARTESIAN_POINT('Ctrl Pts',(21.2393785441268,18.6776565472299,-3.79334189038521));
#50608=CARTESIAN_POINT('Ctrl Pts',(21.21952276158,18.5917164663179,-3.79772835239678));
#50609=CARTESIAN_POINT('Ctrl Pts',(21.1953413592831,18.5071543400131,-3.80211481440834));
#50610=CARTESIAN_POINT('Ctrl Pts',(21.1711599569862,18.4225922137084,-3.80650127641991));
#50611=CARTESIAN_POINT('Ctrl Pts',(21.1426531949957,18.3394085662324,-3.81088773843147));
#50612=CARTESIAN_POINT('Ctrl Pts',(21.1100276507034,18.2580610706384,-3.81527420044303));
#50613=CARTESIAN_POINT('Ctrl Pts',(21.0789032560606,18.1804564938874,-3.81945883483597));
#50614=CARTESIAN_POINT('Ctrl Pts',(21.0439149217344,18.104233954906,-3.82364346922891));
#50615=CARTESIAN_POINT('Ctrl Pts',(21.0052063614281,18.0298049848529,-3.82782810362184));
#50616=CARTESIAN_POINT('Ctrl Pts',(20.9665528979663,17.9554819552262,-3.83200678170567));
#50617=CARTESIAN_POINT('Ctrl Pts',(20.924189937065,17.8829478282645,-3.8361854597895));
#50618=CARTESIAN_POINT('Ctrl Pts',(20.8783095486356,17.8125949944204,-3.84036413787333));
#50619=CARTESIAN_POINT('Ctrl Pts',(20.8316067872157,17.7409811365889,-3.8446177157588));
#50620=CARTESIAN_POINT('Ctrl Pts',(20.7812594376514,17.6716279878893,-3.84887129364426));
#50621=CARTESIAN_POINT('Ctrl Pts',(20.7275195051817,17.6049240421262,-3.85312487152973));
#50622=CARTESIAN_POINT('Ctrl Pts',(20.6748214261695,17.5395132825159,-3.85729598550756));
#50623=CARTESIAN_POINT('Ctrl Pts',(20.6188614359627,17.476650297294,-3.8614670994854));
#50624=CARTESIAN_POINT('Ctrl Pts',(20.5599202972605,17.4166714158069,-3.86563821346324));
#50625=CARTESIAN_POINT('Ctrl Pts',(20.5009989368265,17.3567126608129,-3.8698079277835));
#50626=CARTESIAN_POINT('Ctrl Pts',(20.4390987367876,17.2996364153551,-3.87397764210375));
#50627=CARTESIAN_POINT('Ctrl Pts',(20.3745386111499,17.2457435115675,-3.87814735642401));
#50628=CARTESIAN_POINT('Ctrl Pts',(20.3099807828387,17.1918525255206,-3.88231692236793));
#50629=CARTESIAN_POINT('Ctrl Pts',(20.2427635708238,17.1411449500712,-3.88648648831186));
#50630=CARTESIAN_POINT('Ctrl Pts',(20.1732393309682,17.0938816404853,-3.89065605425579));
#50631=CARTESIAN_POINT('Ctrl Pts',(20.1012707046023,17.0449566112369,-3.89497221699484));
#50632=CARTESIAN_POINT('Ctrl Pts',(20.0268302379304,16.9997228515222,-3.8992883797339));
#50633=CARTESIAN_POINT('Ctrl Pts',(19.9503401869381,16.9584200236974,-3.90360454247296));
#50634=CARTESIAN_POINT('Ctrl Pts',(19.8763417913159,16.9184626311471,-3.90778010666452));
#50635=CARTESIAN_POINT('Ctrl Pts',(19.8004257365565,16.882184163653,-3.91195567085608));
#50636=CARTESIAN_POINT('Ctrl Pts',(19.7229964759442,16.8497533016286,-3.91613123504764));
#50637=CARTESIAN_POINT('Ctrl Pts',(19.6416564474417,16.8156844338573,-3.92051769706044));
#50638=CARTESIAN_POINT('Ctrl Pts',(19.5586468811865,16.7858622689059,-3.92490415907325));
#50639=CARTESIAN_POINT('Ctrl Pts',(19.4744545807604,16.7604231263168,-3.92929062108606));
#50640=CARTESIAN_POINT('Ctrl Pts',(19.3902622803344,16.7349839837277,-3.93367708309886));
#50641=CARTESIAN_POINT('Ctrl Pts',(19.3048878272885,16.7139279285856,-3.93806354511167));
#50642=CARTESIAN_POINT('Ctrl Pts',(19.2188278686569,16.6973289917387,-3.94245000712447));
#50643=CARTESIAN_POINT('Ctrl Pts',(19.1367276562993,16.6814937965827,-3.94663464151747));
#50644=CARTESIAN_POINT('Ctrl Pts',(19.0536980417284,16.6696556340513,-3.95081927591047));
#50645=CARTESIAN_POINT('Ctrl Pts',(18.9701628470245,16.6619164176737,-3.95500391030348));
#50646=CARTESIAN_POINT('Ctrl Pts',(18.8867465543309,16.6541882171128,-3.95918258838736));
#50647=CARTESIAN_POINT('Ctrl Pts',(18.8028265650706,16.6505474159413,-3.96336126647125));
#50648=CARTESIAN_POINT('Ctrl Pts',(18.7188367813175,16.651044907269,-3.96753994455514));
#50649=CARTESIAN_POINT('Ctrl Pts',(18.6333415410517,16.6515513157713,-3.97179352244059));
#50650=CARTESIAN_POINT('Ctrl Pts',(18.5477744529634,16.6563459251098,-3.97604710032604));
#50651=CARTESIAN_POINT('Ctrl Pts',(18.4625985845179,16.6654271230872,-3.98030067821149));
#50652=CARTESIAN_POINT('Ctrl Pts',(18.3790740164904,16.6743322643211,-3.98447179218939));
#50653=CARTESIAN_POINT('Ctrl Pts',(18.2959261128669,16.6873592186152,-3.98864290616729));
#50654=CARTESIAN_POINT('Ctrl Pts',(18.2135896449265,16.7044539576676,-3.9928140201452));
#50655=CARTESIAN_POINT('Ctrl Pts',(18.1312808057832,16.7215429604151,-3.99698373446551));
#50656=CARTESIAN_POINT('Ctrl Pts',(18.049783311613,16.7426969435999,-4.00115344878583));
#50657=CARTESIAN_POINT('Ctrl Pts',(17.9695227367355,16.7678105857401,-4.00532316310615));
#50658=CARTESIAN_POINT('Ctrl Pts',(17.8892650178734,16.7929233342292,-4.00949272905015));
#50659=CARTESIAN_POINT('Ctrl Pts',(17.8102445695787,16.8219953233349,-4.01366229499415));
#50660=CARTESIAN_POINT('Ctrl Pts',(17.7328714533942,16.8548714735458,-4.01783186093816));
#50661=CARTESIAN_POINT('Ctrl Pts',(17.652777993893,16.8889035086419,-4.02214802367714));
#50662=CARTESIAN_POINT('Ctrl Pts',(17.5744503476379,16.9270119844461,-4.02646418641611));
#50663=CARTESIAN_POINT('Ctrl Pts',(17.4983185918994,16.9689715751859,-4.03078034915509));
#50664=CARTESIAN_POINT('Ctrl Pts',(17.4246668200984,17.0095643366696,-4.03495591334672));
#50665=CARTESIAN_POINT('Ctrl Pts',(17.3530704495475,17.0537608783684,-4.03913147753835));
#50666=CARTESIAN_POINT('Ctrl Pts',(17.2838902366718,17.1013124225847,-4.04330704172998));
#50667=CARTESIAN_POINT('Ctrl Pts',(17.2112158957014,17.1512656822582,-4.04769350374263));
#50668=CARTESIAN_POINT('Ctrl Pts',(17.1412086706269,17.2049214186627,-4.05207996575528));
#50669=CARTESIAN_POINT('Ctrl Pts',(17.0742466821561,17.2619440942071,-4.05646642776794));
#50670=CARTESIAN_POINT('Ctrl Pts',(17.0072846936854,17.3189667697514,-4.06085288978059));
#50671=CARTESIAN_POINT('Ctrl Pts',(16.9433683113269,17.3793559306723,-4.06523935179324));
#50672=CARTESIAN_POINT('Ctrl Pts',(16.8828286089282,17.4427340469043,-4.06962581380589));
#50673=CARTESIAN_POINT('Ctrl Pts',(16.8258191500137,17.5024164036099,-4.07375648865202));
#50674=CARTESIAN_POINT('Ctrl Pts',(16.7715797255597,17.5649836670307,-4.07788716349815));
#50675=CARTESIAN_POINT('Ctrl Pts',(16.720421868205,17.6301448177784,-4.08201783834428));
#50676=CARTESIAN_POINT('Ctrl Pts',(16.6693300782615,17.6952218166721,-4.08614317866297));
#50677=CARTESIAN_POINT('Ctrl Pts',(16.6213122506322,17.7628856907896,-4.09026851898165));
#50678=CARTESIAN_POINT('Ctrl Pts',(16.5766430483354,17.8328088002369,-4.09439385930034));
#50679=CARTESIAN_POINT('Ctrl Pts',(16.5320173182039,17.9026638603613,-4.09851518482882));
#50680=CARTESIAN_POINT('Ctrl Pts',(16.4907340001792,17.9747733973529,-4.10263651035731));
#50681=CARTESIAN_POINT('Ctrl Pts',(16.4530264539488,18.0487781269419,-4.10675783588579));
#50682=CARTESIAN_POINT('Ctrl Pts',(16.4153436115609,18.1227343728356,-4.11087646135587));
#50683=CARTESIAN_POINT('Ctrl Pts',(16.3812321043788,18.1985829265154,-4.11499508682596));
#50684=CARTESIAN_POINT('Ctrl Pts',(16.350880245421,18.2759383788566,-4.11911371229604));
#50685=CARTESIAN_POINT('Ctrl Pts',(16.3205285952524,18.3532932990729,-4.12323230943428));
#50686=CARTESIAN_POINT('Ctrl Pts',(16.293936732308,18.4321546644583,-4.12735090657251));
#50687=CARTESIAN_POINT('Ctrl Pts',(16.271245067881,18.5121165016089,-4.13146950371074));
#50688=CARTESIAN_POINT('Ctrl Pts',(16.2485547151171,18.592073716666,-4.13558786277865));
#50689=CARTESIAN_POINT('Ctrl Pts',(16.2297642345969,18.6731308198829,-4.13970622184656));
#50690=CARTESIAN_POINT('Ctrl Pts',(16.2149637529306,18.7548680169618,-4.14382458091447));
#50691=CARTESIAN_POINT('Ctrl Pts',(16.2001500672814,18.8366781344071,-4.14794661410215));
#50692=CARTESIAN_POINT('Ctrl Pts',(16.1893335672673,18.9191690901925,-4.15206864728983));
#50693=CARTESIAN_POINT('Ctrl Pts',(16.1825528364003,19.0019130052847,-4.15619068047751));
#50694=CARTESIAN_POINT('Ctrl Pts',(16.1767848147302,19.0722990307275,-4.15969708372784));
#50695=CARTESIAN_POINT('Ctrl Pts',(16.1739362156169,19.1428678239494,-4.16320348697818));
#50696=CARTESIAN_POINT('Ctrl Pts',(16.1740010840393,19.2133559031925,-4.16670989022851));
#50697=CARTESIAN_POINT('Origin',(18.734,19.211,1.76670989022852));
#50698=CARTESIAN_POINT('',(20.2912843055177,21.2382340775644,-2.85017128750281));
#50699=CARTESIAN_POINT('',(20.2935358855687,21.2411349269503,-2.91665631135199));
#50700=CARTESIAN_POINT('',(20.2935358855687,21.2411349269503,1.76670989022852));
#50701=CARTESIAN_POINT('',(16.1740000028035,19.2108801919503,-3.43329010980363));
#50702=CARTESIAN_POINT('Ctrl Pts',(20.2935358855687,21.2411349269503,-2.91665631135199));
#50703=CARTESIAN_POINT('Ctrl Pts',(20.3304359409714,21.2127885545905,-2.91898054016294));
#50704=CARTESIAN_POINT('Ctrl Pts',(20.3665290680521,21.1834618031319,-2.9213047689739));
#50705=CARTESIAN_POINT('Ctrl Pts',(20.401762322946,21.1532072068041,-2.92362899778486));
#50706=CARTESIAN_POINT('Ctrl Pts',(20.4651976823984,21.0987356230994,-2.92781363217407));
#50707=CARTESIAN_POINT('Ctrl Pts',(20.5260796023552,21.0410515629438,-2.93199826656328));
#50708=CARTESIAN_POINT('Ctrl Pts',(20.5840648143939,20.9804236865549,-2.93618290095248));
#50709=CARTESIAN_POINT('Ctrl Pts',(20.6419674916593,20.919882106445,-2.94036157903251));
#50710=CARTESIAN_POINT('Ctrl Pts',(20.6969813355446,20.8564053626881,-2.94454025711254));
#50711=CARTESIAN_POINT('Ctrl Pts',(20.7487967797138,20.7903017243246,-2.94871893519257));
#50712=CARTESIAN_POINT('Ctrl Pts',(20.8015409785421,20.723013225673,-2.95297251307897));
#50713=CARTESIAN_POINT('Ctrl Pts',(20.8509706214137,20.6530030460431,-2.95722609096538));
#50714=CARTESIAN_POINT('Ctrl Pts',(20.8967991444563,20.5806349370322,-2.96147966885178));
#50715=CARTESIAN_POINT('Ctrl Pts',(20.9417391920986,20.5096698251147,-2.96565078282566));
#50716=CARTESIAN_POINT('Ctrl Pts',(20.9832162459024,20.4364378006298,-2.96982189679954));
#50717=CARTESIAN_POINT('Ctrl Pts',(21.021002390723,20.361313029061,-2.97399301077341));
#50718=CARTESIAN_POINT('Ctrl Pts',(21.0587758560373,20.2862134663357,-2.97816272508966));
#50719=CARTESIAN_POINT('Ctrl Pts',(21.0928606655495,20.2092228285369,-2.98233243940591));
#50720=CARTESIAN_POINT('Ctrl Pts',(21.1230748017628,20.1307399586743,-2.98650215372216));
#50721=CARTESIAN_POINT('Ctrl Pts',(21.153287862827,20.0522598815699,-2.99067171966203));
#50722=CARTESIAN_POINT('Ctrl Pts',(21.1796303599629,19.9722881076019,-2.9948412856019));
#50723=CARTESIAN_POINT('Ctrl Pts',(21.2019688964371,19.8912422555377,-2.99901085154177));
#50724=CARTESIAN_POINT('Ctrl Pts',(21.2250928283449,19.8073469311187,-3.00332701428548));
#50725=CARTESIAN_POINT('Ctrl Pts',(21.2439258622492,19.7223011025982,-3.00764317702919));
#50726=CARTESIAN_POINT('Ctrl Pts',(21.2583771885885,19.6365817309687,-3.0119593397729));
#50727=CARTESIAN_POINT('Ctrl Pts',(21.2723577644625,19.5536546590301,-3.01613490396034));
#50728=CARTESIAN_POINT('Ctrl Pts',(21.2822377087348,19.4700977247691,-3.02031046814778));
#50729=CARTESIAN_POINT('Ctrl Pts',(21.2879876706469,19.3863481627602,-3.02448603233522));
#50730=CARTESIAN_POINT('Ctrl Pts',(21.294028049485,19.2983686091941,-3.02887249435706));
#50731=CARTESIAN_POINT('Ctrl Pts',(21.295510260803,19.2101770410252,-3.03325895637891));
#50732=CARTESIAN_POINT('Ctrl Pts',(21.2924621252161,19.1222782223196,-3.03764541840075));
#50733=CARTESIAN_POINT('Ctrl Pts',(21.2894139896292,19.034379403614,-3.0420318804226));
#50734=CARTESIAN_POINT('Ctrl Pts',(21.2818356329245,18.9467739058741,-3.04641834244444));
#50735=CARTESIAN_POINT('Ctrl Pts',(21.2698170137414,18.859955739515,-3.05080480446629));
#50736=CARTESIAN_POINT('Ctrl Pts',(21.2583513890591,18.7771322058033,-3.05498943886226));
#50737=CARTESIAN_POINT('Ctrl Pts',(21.2428024516836,18.6947168580505,-3.05917407325823));
#50738=CARTESIAN_POINT('Ctrl Pts',(21.2232102976567,18.6131437513584,-3.0633587076542));
#50739=CARTESIAN_POINT('Ctrl Pts',(21.2036460306358,18.531686753886,-3.06753738574111));
#50740=CARTESIAN_POINT('Ctrl Pts',(21.1800500847572,18.4510700597147,-3.07171606382802));
#50741=CARTESIAN_POINT('Ctrl Pts',(21.1525141031145,18.371720825329,-3.07589474191492));
#50742=CARTESIAN_POINT('Ctrl Pts',(21.1244845588153,18.2909493130154,-3.08014831979962));
#50743=CARTESIAN_POINT('Ctrl Pts',(21.09237240526,18.2114916234332,-3.08440189768432));
#50744=CARTESIAN_POINT('Ctrl Pts',(21.0563283883888,18.133785603288,-3.08865547556902));
#50745=CARTESIAN_POINT('Ctrl Pts',(21.0209831550868,18.0575860659054,-3.09282658955002));
#50746=CARTESIAN_POINT('Ctrl Pts',(20.9818573541681,17.9830713215426,-3.09699770353101));
#50747=CARTESIAN_POINT('Ctrl Pts',(20.9391422334475,17.9106355394482,-3.10116881751201));
#50748=CARTESIAN_POINT('Ctrl Pts',(20.896441446198,17.8382240638797,-3.10533853183544));
#50749=CARTESIAN_POINT('Ctrl Pts',(20.8501539646469,17.7678905610384,-3.10950824615888));
#50750=CARTESIAN_POINT('Ctrl Pts',(20.8005166300296,17.7000039649916,-3.11367796048232));
#50751=CARTESIAN_POINT('Ctrl Pts',(20.7508810617214,17.6321197846409,-3.11784752642945));
#50752=CARTESIAN_POINT('Ctrl Pts',(20.697896149566,17.5666827088149,-3.12201709237658));
#50753=CARTESIAN_POINT('Ctrl Pts',(20.6418408397364,17.5040309521746,-3.1261866583237));
#50754=CARTESIAN_POINT('Ctrl Pts',(20.583814694456,17.4391764371619,-3.13050282105904));
#50755=CARTESIAN_POINT('Ctrl Pts',(20.5224985756088,17.3773071422623,-3.13481898379437));
#50756=CARTESIAN_POINT('Ctrl Pts',(20.4582443784125,17.3187575938816,-3.13913514652971));
#50757=CARTESIAN_POINT('Ctrl Pts',(20.3960832548338,17.262115290792,-3.14331071072449));
#50758=CARTESIAN_POINT('Ctrl Pts',(20.3311729226017,17.2085800374226,-3.14748627491927));
#50759=CARTESIAN_POINT('Ctrl Pts',(20.2638651397918,17.1584131798996,-3.15166183911405));
#50760=CARTESIAN_POINT('Ctrl Pts',(20.1931578010453,17.1057125137858,-3.15604830111966));
#50761=CARTESIAN_POINT('Ctrl Pts',(20.1198049419668,17.0567297856998,-3.16043476312527));
#50762=CARTESIAN_POINT('Ctrl Pts',(20.0442460480199,17.0117148221187,-3.16482122513089));
#50763=CARTESIAN_POINT('Ctrl Pts',(19.9686871540731,16.9666998585377,-3.1692076871365));
#50764=CARTESIAN_POINT('Ctrl Pts',(19.8909227738875,16.9256528630382,-3.17359414914211));
#50765=CARTESIAN_POINT('Ctrl Pts',(19.8114169849418,16.8887655931067,-3.17798061114772));
#50766=CARTESIAN_POINT('Ctrl Pts',(19.7355693750926,16.8535755610944,-3.18216524554016));
#50767=CARTESIAN_POINT('Ctrl Pts',(19.6578547653245,16.8220398921686,-3.1863498799326));
#50768=CARTESIAN_POINT('Ctrl Pts',(19.5786598305131,16.7943598176978,-3.19053451432504));
#50769=CARTESIAN_POINT('Ctrl Pts',(19.499577619889,16.7667191423869,-3.19471319240838));
#50770=CARTESIAN_POINT('Ctrl Pts',(19.4190197000616,16.7429233111999,-3.19889187049171));
#50771=CARTESIAN_POINT('Ctrl Pts',(19.3373948467028,16.7231264785017,-3.20307054857505));
#50772=CARTESIAN_POINT('Ctrl Pts',(19.2543069264952,16.7029748018014,-3.20732412646064));
#50773=CARTESIAN_POINT('Ctrl Pts',(19.1701138843273,16.6869671007256,-3.21157770434623));
#50774=CARTESIAN_POINT('Ctrl Pts',(19.0852654759065,16.6752136199127,-3.21583128223181));
#50775=CARTESIAN_POINT('Ctrl Pts',(19.0020620194662,16.6636880032626,-3.22000239620915));
#50776=CARTESIAN_POINT('Ctrl Pts',(18.9182288577836,16.6562531921902,-3.22417351018649));
#50777=CARTESIAN_POINT('Ctrl Pts',(18.8342009436322,16.6529617338876,-3.22834462416383));
#50778=CARTESIAN_POINT('Ctrl Pts',(18.7502012258589,16.6496713800656,-3.23251433848359));
#50779=CARTESIAN_POINT('Ctrl Pts',(18.666007344703,16.6505216357631,-3.23668405280335));
#50780=CARTESIAN_POINT('Ctrl Pts',(18.5820577129978,16.6555130519957,-3.24085376712311));
#50781=CARTESIAN_POINT('Ctrl Pts',(18.4981110685807,16.6605042906122,-3.24502333306655));
#50782=CARTESIAN_POINT('Ctrl Pts',(18.4144091155048,16.6696363686189,-3.24919289900998));
#50783=CARTESIAN_POINT('Ctrl Pts',(18.3313872270485,16.6828578056098,-3.25336246495341));
#50784=CARTESIAN_POINT('Ctrl Pts',(18.2454463913857,16.6965440920191,-3.25767862769306));
#50785=CARTESIAN_POINT('Ctrl Pts',(18.1602348531238,16.7146125685865,-3.2619947904327));
#50786=CARTESIAN_POINT('Ctrl Pts',(18.0762243702396,16.7369484199206,-3.26631095317235));
#50787=CARTESIAN_POINT('Ctrl Pts',(17.9949505200243,16.7585566832401,-3.27048651736343));
#50788=CARTESIAN_POINT('Ctrl Pts',(17.9148011124186,16.784158383043,-3.27466208155451));
#50789=CARTESIAN_POINT('Ctrl Pts',(17.8361862981298,16.813599208156,-3.27883764574559));
#50790=CARTESIAN_POINT('Ctrl Pts',(17.7536008364222,16.8445270193708,-3.28322410775951));
#50791=CARTESIAN_POINT('Ctrl Pts',(17.6727096022458,16.8796917438774,-3.28761056977344));
#50792=CARTESIAN_POINT('Ctrl Pts',(17.5939605452813,16.9188590702828,-3.29199703178737));
#50793=CARTESIAN_POINT('Ctrl Pts',(17.5152114883168,16.9580263966883,-3.2963834938013));
#50794=CARTESIAN_POINT('Ctrl Pts',(17.4386050767024,17.001195973874,-3.30076995581523));
#50795=CARTESIAN_POINT('Ctrl Pts',(17.364553744478,17.0480813808105,-3.30515641782915));
#50796=CARTESIAN_POINT('Ctrl Pts',(17.2939096238495,17.092809520654,-3.30934105222176));
#50797=CARTESIAN_POINT('Ctrl Pts',(17.2253276726157,17.1410855493988,-3.31352568661436));
#50798=CARTESIAN_POINT('Ctrl Pts',(17.1591863942882,17.19269325739,-3.31771032100696));
#50799=CARTESIAN_POINT('Ctrl Pts',(17.0931392598839,17.2442275081965,-3.32188899909045));
#50800=CARTESIAN_POINT('Ctrl Pts',(17.0295262575255,17.2990837381083,-3.32606767717394));
#50801=CARTESIAN_POINT('Ctrl Pts',(16.9686982691563,17.3570016723092,-3.33024635525743));
#50802=CARTESIAN_POINT('Ctrl Pts',(16.9067799828036,17.4159577438638,-3.33449993314298));
#50803=CARTESIAN_POINT('Ctrl Pts',(16.8477479425957,17.4780861035064,-3.33875351102853));
#50804=CARTESIAN_POINT('Ctrl Pts',(16.7919382910611,17.5430682511945,-3.34300708891407));
#50805=CARTESIAN_POINT('Ctrl Pts',(16.7372106185328,17.6067905931384,-3.34717820289155));
#50806=CARTESIAN_POINT('Ctrl Pts',(16.6855818186072,17.6732566930094,-3.35134931686903));
#50807=CARTESIAN_POINT('Ctrl Pts',(16.6373315068437,17.742129267156,-3.35552043084651));
#50808=CARTESIAN_POINT('Ctrl Pts',(16.5890973859384,17.810978730445,-3.3596901451664));
#50809=CARTESIAN_POINT('Ctrl Pts',(16.5442397654171,17.8822326878121,-3.36385985948629));
#50810=CARTESIAN_POINT('Ctrl Pts',(16.5029964131481,17.9555228016989,-3.36802957380618));
#50811=CARTESIAN_POINT('Ctrl Pts',(16.4617545284947,18.0288103076089,-3.37219913974973));
#50812=CARTESIAN_POINT('Ctrl Pts',(16.4241268812486,18.1041334246491,-3.37636870569329));
#50813=CARTESIAN_POINT('Ctrl Pts',(16.3903058438335,18.1810982074242,-3.38053827163684));
#50814=CARTESIAN_POINT('Ctrl Pts',(16.3552957004569,18.2607689770351,-3.38485443437632));
#50815=CARTESIAN_POINT('Ctrl Pts',(16.3243650403573,18.3421985193633,-3.3891705971158));
#50816=CARTESIAN_POINT('Ctrl Pts',(16.2976726756056,18.4249280132142,-3.39348675985528));
#50817=CARTESIAN_POINT('Ctrl Pts',(16.2718498118346,18.5049626024846,-3.39766232404646));
#50818=CARTESIAN_POINT('Ctrl Pts',(16.2499934356292,18.5862132848944,-3.40183788823764));
#50819=CARTESIAN_POINT('Ctrl Pts',(16.2321958025117,18.6682516628952,-3.40601345242882));
#50820=CARTESIAN_POINT('Ctrl Pts',(16.2134992532484,18.7544336043728,-3.41039991444245));
#50821=CARTESIAN_POINT('Ctrl Pts',(16.1992823307861,18.8414843294194,-3.41478637645608));
#50822=CARTESIAN_POINT('Ctrl Pts',(16.1895904829899,18.9289003549305,-3.41917283846971));
#50823=CARTESIAN_POINT('Ctrl Pts',(16.1798986351937,19.0163163804415,-3.42355930048334));
#50824=CARTESIAN_POINT('Ctrl Pts',(16.174731820223,19.1040971227329,-3.42794576249697));
#50825=CARTESIAN_POINT('Ctrl Pts',(16.1740724460423,19.1917407557755,-3.43233222451059));
#50826=CARTESIAN_POINT('Ctrl Pts',(16.1740244495167,19.1981204260764,-3.43265151959756));
#50827=CARTESIAN_POINT('Ctrl Pts',(16.1740003013853,19.204500276023,-3.43297081468453));
#50828=CARTESIAN_POINT('Ctrl Pts',(16.1740000028035,19.2108801913083,-3.4332901097715));
#50829=CARTESIAN_POINT('Ctrl Pts',(16.1740000028035,19.2108801919503,-3.43329010980363));
#50830=CARTESIAN_POINT('Ctrl Pts',(16.173996094898,19.2943824116246,-3.43746913841142));
#50831=CARTESIAN_POINT('Ctrl Pts',(16.1780820066338,19.3780422026732,-3.4416481670192));
#50832=CARTESIAN_POINT('Ctrl Pts',(16.1862780259001,19.4614251239166,-3.44582719562699));
#50833=CARTESIAN_POINT('Ctrl Pts',(16.1944623792895,19.5446893613378,-3.45000027597725));
#50834=CARTESIAN_POINT('Ctrl Pts',(16.2067451760218,19.6276770564327,-3.45417335632751));
#50835=CARTESIAN_POINT('Ctrl Pts',(16.2230946976723,19.7099534675123,-3.45834643667778));
#50836=CARTESIAN_POINT('Ctrl Pts',(16.2396087147061,19.7930576758859,-3.46256150311587));
#50837=CARTESIAN_POINT('Ctrl Pts',(16.2602717621694,19.8754357285734,-3.46677656955397));
#50838=CARTESIAN_POINT('Ctrl Pts',(16.2849973159137,19.9566445891563,-3.47099163599206));
#50839=CARTESIAN_POINT('Ctrl Pts',(16.3094325809408,20.0369000225196,-3.47515721572334));
#50840=CARTESIAN_POINT('Ctrl Pts',(16.3378353258574,20.1160131199902,-3.47932279545462));
#50841=CARTESIAN_POINT('Ctrl Pts',(16.3700710228283,20.1935679573893,-3.4834883751859));
#50842=CARTESIAN_POINT('Ctrl Pts',(16.4022960455082,20.2710971138511,-3.48765257555782));
#50843=CARTESIAN_POINT('Ctrl Pts',(16.4383513227395,20.3470686092118,-3.49181677592973));
#50844=CARTESIAN_POINT('Ctrl Pts',(16.4780536821042,20.4210852080628,-3.49598097630165));
#50845=CARTESIAN_POINT('Ctrl Pts',(16.5177548909312,20.495099661981,-3.50014505599888));
#50846=CARTESIAN_POINT('Ctrl Pts',(16.561102752779,20.5671589258651,-3.50430913569611));
#50847=CARTESIAN_POINT('Ctrl Pts',(16.6078681568273,20.636890383391,-3.50847321539335));
#50848=CARTESIAN_POINT('Ctrl Pts',(16.6556310871523,20.7081092430383,-3.5127261167099));
#50849=CARTESIAN_POINT('Ctrl Pts',(16.7069587733461,20.7768994173764,-3.51697901802646));
#50850=CARTESIAN_POINT('Ctrl Pts',(16.761561649075,20.8428967344168,-3.52123191934301));
#50851=CARTESIAN_POINT('Ctrl Pts',(16.8151012611779,20.9076089076679,-3.52540200532769));
#50852=CARTESIAN_POINT('Ctrl Pts',(16.8717892886061,20.9696357146529,-3.52957209131237));
#50853=CARTESIAN_POINT('Ctrl Pts',(16.9313144499797,21.028670159228,-3.53374217729704));
#50854=CARTESIAN_POINT('Ctrl Pts',(16.9926128107595,21.0894631852106,-3.53803648627954));
#50855=CARTESIAN_POINT('Ctrl Pts',(17.0569196193486,21.1470823903912,-3.54233079526204));
#50856=CARTESIAN_POINT('Ctrl Pts',(17.1238587796064,21.2012374859271,-3.54662510424453));
#50857=CARTESIAN_POINT('Ctrl Pts',(17.1907979398641,21.255392581463,-3.55091941322703));
#50858=CARTESIAN_POINT('Ctrl Pts',(17.2603689845985,21.3060833143331,-3.55521372220952));
#50859=CARTESIAN_POINT('Ctrl Pts',(17.3321657913456,21.3530692919339,-3.55950803119202));
#50860=CARTESIAN_POINT('Ctrl Pts',(17.4021289421207,21.3988552702266,-3.56369266558496));
#50861=CARTESIAN_POINT('Ctrl Pts',(17.4744678068902,21.4412951999105,-3.5678772999779));
#50862=CARTESIAN_POINT('Ctrl Pts',(17.5488288662329,21.4801340603158,-3.57206193437084));
#50863=CARTESIAN_POINT('Ctrl Pts',(17.6230840818118,21.5189176384105,-3.57624061245467));
#50864=CARTESIAN_POINT('Ctrl Pts',(17.6993553703912,21.5541101172787,-3.58041929053851));
#50865=CARTESIAN_POINT('Ctrl Pts',(17.7772605377966,21.5854998634371,-3.58459796862235));
#50866=CARTESIAN_POINT('Ctrl Pts',(17.8565620993408,21.6174522482369,-3.58885154650781));
#50867=CARTESIAN_POINT('Ctrl Pts',(17.9375562869758,21.6454639674282,-3.59310512439327));
#50868=CARTESIAN_POINT('Ctrl Pts',(18.0198140087909,21.6693609112497,-3.59735870227874));
#50869=CARTESIAN_POINT('Ctrl Pts',(18.1004770041531,21.6927945661834,-3.60152981625657));
#50870=CARTESIAN_POINT('Ctrl Pts',(18.1823545166283,21.7122714336376,-3.60570093023441));
#50871=CARTESIAN_POINT('Ctrl Pts',(18.265023760118,21.7276766352526,-3.60987204421225));
#50872=CARTESIAN_POINT('Ctrl Pts',(18.3476652631446,21.7430766675033,-3.6140417585325));
#50873=CARTESIAN_POINT('Ctrl Pts',(18.4310975176837,21.754407663177,-3.61821147285276));
#50874=CARTESIAN_POINT('Ctrl Pts',(18.5148867965887,21.7616056935737,-3.62238118717302));
#50875=CARTESIAN_POINT('Ctrl Pts',(18.5986730939115,21.7688034678337,-3.62655075311694));
#50876=CARTESIAN_POINT('Ctrl Pts',(18.6828159319229,21.7718685307012,-3.63072031906087));
#50877=CARTESIAN_POINT('Ctrl Pts',(18.7668770686622,21.7707888776921,-3.63488988500479));
#50878=CARTESIAN_POINT('Ctrl Pts',(18.8538936912738,21.7696712654151,-3.63920604774385));
#50879=CARTESIAN_POINT('Ctrl Pts',(18.9408222331037,21.764112064791,-3.6435222104829));
#50880=CARTESIAN_POINT('Ctrl Pts',(19.0271792931092,21.7541566806023,-3.64783837322196));
#50881=CARTESIAN_POINT('Ctrl Pts',(19.1107232809632,21.744525592007,-3.65201393741352));
#50882=CARTESIAN_POINT('Ctrl Pts',(19.193731990268,21.7307804563761,-3.65618950160509));
#50883=CARTESIAN_POINT('Ctrl Pts',(19.2757772698984,21.7130146661883,-3.66036506579665));
#50884=CARTESIAN_POINT('Ctrl Pts',(19.3619664615664,21.6943515681707,-3.66475152780945));
#50885=CARTESIAN_POINT('Ctrl Pts',(19.4470917766263,21.6712511277377,-3.66913798982225));
#50886=CARTESIAN_POINT('Ctrl Pts',(19.5306760960808,21.6438804323134,-3.67352445183505));
#50887=CARTESIAN_POINT('Ctrl Pts',(19.6142604155353,21.6165097368891,-3.67791091384786));
#50888=CARTESIAN_POINT('Ctrl Pts',(19.6963032254016,21.584869066222,-3.68229737586066));
#50889=CARTESIAN_POINT('Ctrl Pts',(19.7763550154477,21.5491822045707,-3.68668383787346));
#50890=CARTESIAN_POINT('Ctrl Pts',(19.8527263004245,21.5151361016724,-3.6908686254994));
#50891=CARTESIAN_POINT('Ctrl Pts',(19.9275699049942,21.4772809673763,-3.69505341312535));
#50892=CARTESIAN_POINT('Ctrl Pts',(20.0004799995006,21.4357760361135,-3.69923820075129));
#50893=CARTESIAN_POINT('Ctrl Pts',(20.0732773467754,21.3943352875421,-3.70341651707552));
#50894=CARTESIAN_POINT('Ctrl Pts',(20.1441467296573,21.3492561841679,-3.70759483339976));
#50895=CARTESIAN_POINT('Ctrl Pts',(20.212703423182,21.3007454836103,-3.71177314972399));
#50896=CARTESIAN_POINT('Ctrl Pts',(20.2400223166183,21.2814146409031,-3.71343815094468));
#50897=CARTESIAN_POINT('Ctrl Pts',(20.2669742248431,21.2615394146186,-3.71510315216536));
#50898=CARTESIAN_POINT('Ctrl Pts',(20.2935358855687,21.2411349269503,-3.71676815338605));
#50899=CARTESIAN_POINT('',(16.174394460606,19.210617605254,-3.3667098651142));
#50900=CARTESIAN_POINT('Ctrl Pts',(16.1740000284928,19.2106180532904,-3.36670989022851));
#50901=CARTESIAN_POINT('Ctrl Pts',(16.1739869935966,19.297984518944,-3.37103154303559));
#50902=CARTESIAN_POINT('Ctrl Pts',(16.1784506871913,19.3852864628672,-3.37535319584266));
#50903=CARTESIAN_POINT('Ctrl Pts',(16.1873453738308,19.472055961455,-3.37967484864974));
#50904=CARTESIAN_POINT('Ctrl Pts',(16.1966194662204,19.5625266412114,-3.38418084296216));
#50905=CARTESIAN_POINT('Ctrl Pts',(16.2107109130556,19.6524179424094,-3.38868683727458));
#50906=CARTESIAN_POINT('Ctrl Pts',(16.2295088315793,19.7412112666689,-3.39319283158699));
#50907=CARTESIAN_POINT('Ctrl Pts',(16.2475982064586,19.8266577339084,-3.39752898296558));
#50908=CARTESIAN_POINT('Ctrl Pts',(16.2700454505064,19.9110871351913,-3.40186513434416));
#50909=CARTESIAN_POINT('Ctrl Pts',(16.2967009964589,19.9940540002691,-3.40620128572275));
#50910=CARTESIAN_POINT('Ctrl Pts',(16.3233900671467,20.0771252129449,-3.41054289068791));
#50911=CARTESIAN_POINT('Ctrl Pts',(16.354297844581,20.1587298407162,-3.41488449565307));
#50912=CARTESIAN_POINT('Ctrl Pts',(16.3892268388774,20.2384428562597,-3.41922610061823));
#50913=CARTESIAN_POINT('Ctrl Pts',(16.4242296046623,20.318324229007,-3.42357687523362));
#50914=CARTESIAN_POINT('Ctrl Pts',(16.4632703651621,20.3963056454692,-3.42792764984902));
#50915=CARTESIAN_POINT('Ctrl Pts',(16.5061059491326,20.4719869539808,-3.43227842446442));
#50916=CARTESIAN_POINT('Ctrl Pts',(16.5109248522386,20.4805009243496,-3.43276787644252));
#50917=CARTESIAN_POINT('Ctrl Pts',(16.5157917376009,20.4889858169829,-3.43325732842063));
#50918=CARTESIAN_POINT('Ctrl Pts',(16.5207062260026,20.4974410868688,-3.43374678039873));
#50919=CARTESIAN_POINT('Ctrl Pts',(16.5627232942887,20.5697305345463,-3.43793141479118));
#50920=CARTESIAN_POINT('Ctrl Pts',(16.608363899273,20.6400938357955,-3.44211604918362));
#50921=CARTESIAN_POINT('Ctrl Pts',(16.6574263400684,20.7081445604478,-3.44630068357607));
#50922=CARTESIAN_POINT('Ctrl Pts',(16.7064189465521,20.7760984233165,-3.4504793616594));
#50923=CARTESIAN_POINT('Ctrl Pts',(16.7588234476462,20.8417458779045,-3.45465803974274));
#50924=CARTESIAN_POINT('Ctrl Pts',(16.8143930615575,20.9047264247462,-3.45883671782608));
#50925=CARTESIAN_POINT('Ctrl Pts',(16.8709587208712,20.9688358526383,-3.46309029571167));
#50926=CARTESIAN_POINT('Ctrl Pts',(16.9308038360938,21.0301814068962,-3.46734387359725));
#50927=CARTESIAN_POINT('Ctrl Pts',(16.9936228831502,21.0884151089052,-3.47159745148284));
#50928=CARTESIAN_POINT('Ctrl Pts',(17.055224060387,21.1455198369568,-3.47576856546018));
#50929=CARTESIAN_POINT('Ctrl Pts',(17.1196845346186,21.1996319675306,-3.47993967943753));
#50930=CARTESIAN_POINT('Ctrl Pts',(17.1866778681087,21.250459296029,-3.48411079341487));
#50931=CARTESIAN_POINT('Ctrl Pts',(17.2536487213387,21.3012695689265,-3.48828050773464));
#50932=CARTESIAN_POINT('Ctrl Pts',(17.3231503796755,21.3487969510058,-3.4924502220544));
#50933=CARTESIAN_POINT('Ctrl Pts',(17.3948237869028,21.3927898776634,-3.49661993637417));
#50934=CARTESIAN_POINT('Ctrl Pts',(17.4664946436827,21.436781238864,-3.50078950231762));
#50935=CARTESIAN_POINT('Ctrl Pts',(17.5403367031862,21.477238154784,-3.50495906826106));
#50936=CARTESIAN_POINT('Ctrl Pts',(17.6159635983352,21.5139534525371,-3.5091286342045));
#50937=CARTESIAN_POINT('Ctrl Pts',(17.6942494418461,21.5519596148778,-3.51344479694414));
#50938=CARTESIAN_POINT('Ctrl Pts',(17.7744474914063,21.5859559226943,-3.51776095968378));
#50939=CARTESIAN_POINT('Ctrl Pts',(17.8561052781564,21.6157662791546,-3.52207712242342));
#50940=CARTESIAN_POINT('Ctrl Pts',(17.9351030710677,21.6446055663799,-3.5262526866145));
#50941=CARTESIAN_POINT('Ctrl Pts',(18.0154664958613,21.6695273345316,-3.53042825080559));
#50942=CARTESIAN_POINT('Ctrl Pts',(18.0967709615466,21.6904231491522,-3.53460381499668));
#50943=CARTESIAN_POINT('Ctrl Pts',(18.1821819225495,21.7123743617041,-3.53899027701059));
#50944=CARTESIAN_POINT('Ctrl Pts',(18.2686309144575,21.7298821146794,-3.5433767390245));
#50945=CARTESIAN_POINT('Ctrl Pts',(18.3556165397336,21.7428819002862,-3.54776320103842));
#50946=CARTESIAN_POINT('Ctrl Pts',(18.4426021650097,21.755881685893,-3.55214966305233));
#50947=CARTESIAN_POINT('Ctrl Pts',(18.5301238388031,21.7643735238079,-3.55653612506624));
#50948=CARTESIAN_POINT('Ctrl Pts',(18.6176794289204,21.7683559636358,-3.56092258708016));
#50949=CARTESIAN_POINT('Ctrl Pts',(18.7011876748678,21.7721543112247,-3.56510628052802));
#50950=CARTESIAN_POINT('Ctrl Pts',(18.7850375342269,21.7718650921499,-3.56928997397588));
#50951=CARTESIAN_POINT('Ctrl Pts',(18.8687951970932,21.7674487585009,-3.57347366742374));
#50952=CARTESIAN_POINT('Ctrl Pts',(18.9524422754805,21.7630382556969,-3.57765183717927));
#50953=CARTESIAN_POINT('Ctrl Pts',(19.0359969440171,21.7545114802047,-3.5818300069348));
#50954=CARTESIAN_POINT('Ctrl Pts',(19.1190226609998,21.7418807855205,-3.58600817669033));
#50955=CARTESIAN_POINT('Ctrl Pts',(19.2019636761051,21.729262976525,-3.59018208392535));
#50956=CARTESIAN_POINT('Ctrl Pts',(19.2843763591294,21.712549632003,-3.59435599116036));
#50957=CARTESIAN_POINT('Ctrl Pts',(19.3658279303823,21.6918050037012,-3.59852989839538));
#50958=CARTESIAN_POINT('Ctrl Pts',(19.4496036345041,21.670468449771,-3.60282290357838));
#50959=CARTESIAN_POINT('Ctrl Pts',(19.532362045609,21.6448670908952,-3.60711590876138));
#50960=CARTESIAN_POINT('Ctrl Pts',(19.613642591816,21.6151274738797,-3.61140891394438));
#50961=CARTESIAN_POINT('Ctrl Pts',(19.692588988533,21.5862418953165,-3.61557863605011));
#50962=CARTESIAN_POINT('Ctrl Pts',(19.770140803741,21.5534527148571,-3.61974835815585));
#50963=CARTESIAN_POINT('Ctrl Pts',(19.845892348409,21.5169261491968,-3.62391808026158));
#50964=CARTESIAN_POINT('Ctrl Pts',(19.9250034275847,21.4787796527704,-3.62827272698321));
#50965=CARTESIAN_POINT('Ctrl Pts',(20.0021503442013,21.4365567646314,-3.63262737370485));
#50966=CARTESIAN_POINT('Ctrl Pts',(20.0768973698964,21.3905014691267,-3.63698202042648));
#50967=CARTESIAN_POINT('Ctrl Pts',(20.1516443955915,21.344446173622,-3.64133666714812));
#50968=CARTESIAN_POINT('Ctrl Pts',(20.2239910581103,21.2945587918557,-3.64569131386975));
#50969=CARTESIAN_POINT('Ctrl Pts',(20.2935358855687,21.2411349269503,-3.65004596059139));
#50970=CARTESIAN_POINT('Ctrl Pts',(20.2912843055177,21.2382340775644,-2.85017128750281));
#50971=CARTESIAN_POINT('Ctrl Pts',(20.6891190168232,20.9296543890738,-2.87512870955954));
#50972=CARTESIAN_POINT('Ctrl Pts',(21.5323502710954,19.7924126903705,-2.94247806717674));
#50973=CARTESIAN_POINT('Ctrl Pts',(21.1037095810087,17.3274479097959,-3.05221936035442));
#50974=CARTESIAN_POINT('Ctrl Pts',(18.4329096216685,16.1989182335261,-3.17939516703586));
#50975=CARTESIAN_POINT('Ctrl Pts',(16.4590845281242,17.5465283070756,-3.28422525531049));
#50976=CARTESIAN_POINT('Ctrl Pts',(16.1776267405031,18.8060181972744,-3.34666340802465));
#50977=CARTESIAN_POINT('Ctrl Pts',(16.1781627672566,19.2106133248248,-3.36670962517832));
#50978=CARTESIAN_POINT('Origin',(18.734,19.211,1.76670989022852));
#50979=CARTESIAN_POINT('',(20.2935358855687,21.2411349269503,-2.05017637612677));
#50980=CARTESIAN_POINT('',(20.2935358855687,21.2411349269503,-2.11663751762489));
#50981=CARTESIAN_POINT('',(20.2935358855687,21.2411349269503,1.76670989022852));
#50982=CARTESIAN_POINT('',(16.1740010149448,19.2132795868243,-2.63329010980609));
#50983=CARTESIAN_POINT('Ctrl Pts',(20.2935358855687,21.2411349269503,-2.11663751762489));
#50984=CARTESIAN_POINT('Ctrl Pts',(20.3602472229086,21.1898877299415,-2.12081218256376));
#50985=CARTESIAN_POINT('Ctrl Pts',(20.424391713608,21.1353781809648,-2.12498684750263));
#50986=CARTESIAN_POINT('Ctrl Pts',(20.485647461214,21.0779041677661,-2.12916151244151));
#50987=CARTESIAN_POINT('Ctrl Pts',(20.5469405618567,21.0203951075881,-2.13333872304211));
#50988=CARTESIAN_POINT('Ctrl Pts',(20.6053410936532,20.9599183157007,-2.13751593364272));
#50989=CARTESIAN_POINT('Ctrl Pts',(20.6605654824905,20.8968070594455,-2.14169314424333));
#50990=CARTESIAN_POINT('Ctrl Pts',(20.7158816120992,20.8335909604667,-2.14587729417872));
#50991=CARTESIAN_POINT('Ctrl Pts',(20.7680107808068,20.7677320210624,-2.15006144411412));
#50992=CARTESIAN_POINT('Ctrl Pts',(20.8167112376172,20.6995946058962,-2.15424559404952));
#50993=CARTESIAN_POINT('Ctrl Pts',(20.8412645276369,20.6652417922813,-2.1563551152651));
#50994=CARTESIAN_POINT('Ctrl Pts',(20.8649469909646,20.6303102486314,-2.15846463648067));
#50995=CARTESIAN_POINT('Ctrl Pts',(20.887732090256,20.5948490103337,-2.16057415769625));
#50996=CARTESIAN_POINT('Ctrl Pts',(20.9329306422986,20.5245049401061,-2.16475879183929));
#50997=CARTESIAN_POINT('Ctrl Pts',(20.9747633711854,20.4518132565708,-2.16894342598234));
#50998=CARTESIAN_POINT('Ctrl Pts',(21.0129782252718,20.3771296020327,-2.17312806012539));
#50999=CARTESIAN_POINT('Ctrl Pts',(21.0511386852002,20.3025522505174,-2.17730673795494));
#51000=CARTESIAN_POINT('Ctrl Pts',(21.0856912912948,20.2259889658803,-2.1814854157845));
#51001=CARTESIAN_POINT('Ctrl Pts',(21.1164276176732,20.1478237008892,-2.18566409361405));
#51002=CARTESIAN_POINT('Ctrl Pts',(21.1477148729807,20.0682573736764,-2.18991767156253));
#51003=CARTESIAN_POINT('Ctrl Pts',(21.1750474280242,19.9870314755984,-2.19417124951102));
#51004=CARTESIAN_POINT('Ctrl Pts',(21.1982547719723,19.9045765414226,-2.1984248274595));
#51005=CARTESIAN_POINT('Ctrl Pts',(21.2210121944984,19.8237201633468,-2.20259594117411));
#51006=CARTESIAN_POINT('Ctrl Pts',(21.2398027993352,19.7416824418443,-2.20676705488871));
#51007=CARTESIAN_POINT('Ctrl Pts',(21.2545152522168,19.658887110043,-2.21093816860331));
#51008=CARTESIAN_POINT('Ctrl Pts',(21.2692227681826,19.5761195610716,-2.21510788265757));
#51009=CARTESIAN_POINT('Ctrl Pts',(21.2798547695701,19.4925953592547,-2.21927759671182));
#51010=CARTESIAN_POINT('Ctrl Pts',(21.2863509615982,19.4087487517752,-2.22344731076607));
#51011=CARTESIAN_POINT('Ctrl Pts',(21.2928469224601,19.3249051279668,-2.22761687644157));
#51012=CARTESIAN_POINT('Ctrl Pts',(21.295207331893,19.2407395800309,-2.23178644211707));
#51013=CARTESIAN_POINT('Ctrl Pts',(21.2934238553146,19.1566904350363,-2.23595600779257));
#51014=CARTESIAN_POINT('Ctrl Pts',(21.2915776736484,19.0696862139404,-2.24027217084133));
#51015=CARTESIAN_POINT('Ctrl Pts',(21.2852907961475,18.9828072608784,-2.24458833389009));
#51016=CARTESIAN_POINT('Ctrl Pts',(21.2746126736334,18.8965365799125,-2.24890449693885));
#51017=CARTESIAN_POINT('Ctrl Pts',(21.2642823912514,18.8130761687308,-2.25308006085863));
#51018=CARTESIAN_POINT('Ctrl Pts',(21.2498426885277,18.730185465086,-2.25725562477842));
#51019=CARTESIAN_POINT('Ctrl Pts',(21.231390539663,18.6482918230543,-2.26143118869821));
#51020=CARTESIAN_POINT('Ctrl Pts',(21.2120064127083,18.562261910464,-2.26581765131146));
#51021=CARTESIAN_POINT('Ctrl Pts',(21.1881940056825,18.4773329923524,-2.2702041139247));
#51022=CARTESIAN_POINT('Ctrl Pts',(21.1601243952751,18.3939807721657,-2.27459057653795));
#51023=CARTESIAN_POINT('Ctrl Pts',(21.1320547848677,18.3106285519789,-2.27897703915119));
#51024=CARTESIAN_POINT('Ctrl Pts',(21.0997282551214,18.2288535413399,-2.28336350176443));
#51025=CARTESIAN_POINT('Ctrl Pts',(21.0633723464423,18.1491033611364,-2.28774996437768));
#51026=CARTESIAN_POINT('Ctrl Pts',(21.0286892306356,18.0730226128866,-2.29193459890683));
#51027=CARTESIAN_POINT('Ctrl Pts',(20.9902102866642,17.9985012713197,-2.29611923343598));
#51028=CARTESIAN_POINT('Ctrl Pts',(20.9480981227546,17.925943774454,-2.30030386796514));
#51029=CARTESIAN_POINT('Ctrl Pts',(20.9060459002788,17.8534895541713,-2.30448254618689));
#51030=CARTESIAN_POINT('Ctrl Pts',(20.8603709589165,17.7829940207375,-2.30866122440865));
#51031=CARTESIAN_POINT('Ctrl Pts',(20.8112833253067,17.7148402537152,-2.3128399026304));
#51032=CARTESIAN_POINT('Ctrl Pts',(20.7613158331932,17.6454648822467,-2.3170934804816));
#51033=CARTESIAN_POINT('Ctrl Pts',(20.7078123007188,17.5785164937711,-2.32134705833279));
#51034=CARTESIAN_POINT('Ctrl Pts',(20.6510424452123,17.5143715011074,-2.32560063618399));
#51035=CARTESIAN_POINT('Ctrl Pts',(20.5953731818021,17.4514700816625,-2.32977175030294));
#51036=CARTESIAN_POINT('Ctrl Pts',(20.5365634319281,17.3912646900244,-2.33394286442189));
#51037=CARTESIAN_POINT('Ctrl Pts',(20.4749092250524,17.3340782994148,-2.33811397854084));
#51038=CARTESIAN_POINT('Ctrl Pts',(20.4132757068275,17.2769110982382,-2.34228369300309));
#51039=CARTESIAN_POINT('Ctrl Pts',(20.3487999642247,17.2227611987298,-2.34645340746534));
#51040=CARTESIAN_POINT('Ctrl Pts',(20.281814494063,17.1719143490357,-2.35062312192759));
#51041=CARTESIAN_POINT('Ctrl Pts',(20.2148314075206,17.1210693086822,-2.35479268801421));
#51042=CARTESIAN_POINT('Ctrl Pts',(20.1453391379229,17.073527361915,-2.35896225410082));
#51043=CARTESIAN_POINT('Ctrl Pts',(20.0737017376934,17.0295327749376,-2.36313182018743));
#51044=CARTESIAN_POINT('Ctrl Pts',(19.9995456602385,16.983991395867,-2.36744798276007));
#51045=CARTESIAN_POINT('Ctrl Pts',(19.9230912497119,16.942251743645,-2.37176414533271));
#51046=CARTESIAN_POINT('Ctrl Pts',(19.8447714026906,16.9045336787708,-2.37608030790535));
#51047=CARTESIAN_POINT('Ctrl Pts',(19.769002810937,16.8680442732384,-2.38025587223989));
#51048=CARTESIAN_POINT('Ctrl Pts',(19.6914889015773,16.8353186124795,-2.38443143657442));
#51049=CARTESIAN_POINT('Ctrl Pts',(19.6126415021214,16.8065064752115,-2.38860700090896));
#51050=CARTESIAN_POINT('Ctrl Pts',(19.5298117168534,16.7762391086339,-2.39299346260065));
#51051=CARTESIAN_POINT('Ctrl Pts',(19.4455107504595,16.7502911703632,-2.39737992429234));
#51052=CARTESIAN_POINT('Ctrl Pts',(19.3602311944416,16.7287763011549,-2.40176638598403));
#51053=CARTESIAN_POINT('Ctrl Pts',(19.2749516384237,16.7072614319465,-2.40615284767573));
#51054=CARTESIAN_POINT('Ctrl Pts',(19.1886940767219,16.6901796698973,-2.41053930936742));
#51055=CARTESIAN_POINT('Ctrl Pts',(19.1019580505852,16.6775819782338,-2.41492577105911));
#51056=CARTESIAN_POINT('Ctrl Pts',(19.0192128717126,16.6655639241852,-2.41911040544303));
#51057=CARTESIAN_POINT('Ctrl Pts',(18.9357242972398,16.6575816378624,-2.42329503982696));
#51058=CARTESIAN_POINT('Ctrl Pts',(18.8519204122534,16.6537173061286,-2.42747967421088));
#51059=CARTESIAN_POINT('Ctrl Pts',(18.7682358117204,16.6498584747926,-2.43165835228591));
#51060=CARTESIAN_POINT('Ctrl Pts',(18.6842372477567,16.6501059764731,-2.43583703036094));
#51061=CARTESIAN_POINT('Ctrl Pts',(18.6003605130588,16.6544905657264,-2.44001570843598));
#51062=CARTESIAN_POINT('Ctrl Pts',(18.5149803479453,16.6589537456027,-2.44426928632367));
#51063=CARTESIAN_POINT('Ctrl Pts',(18.4297268997696,16.6677038557791,-2.44852286421136));
#51064=CARTESIAN_POINT('Ctrl Pts',(18.3450626650525,16.6807178518031,-2.45277644209905));
#51065=CARTESIAN_POINT('Ctrl Pts',(18.2620398119428,16.6934795460874,-2.45694755606873));
#51066=CARTESIAN_POINT('Ctrl Pts',(18.1795840056908,16.7103412009465,-2.4611186700384));
#51067=CARTESIAN_POINT('Ctrl Pts',(18.0981270507742,16.7312287217481,-2.46528978400808));
#51068=CARTESIAN_POINT('Ctrl Pts',(18.0166974295208,16.7521092335416,-2.46945949832043));
#51069=CARTESIAN_POINT('Ctrl Pts',(17.9362664391865,16.7770128141616,-2.47362921263277));
#51070=CARTESIAN_POINT('Ctrl Pts',(17.8572543229417,16.8058145564719,-2.47779892694511));
#51071=CARTESIAN_POINT('Ctrl Pts',(17.7782450182819,16.8346152738944,-2.4819684928814));
#51072=CARTESIAN_POINT('Ctrl Pts',(17.7006549192462,16.8673137188579,-2.48613805881768));
#51073=CARTESIAN_POINT('Ctrl Pts',(17.6248864697071,16.9037359975674,-2.49030762475396));
#51074=CARTESIAN_POINT('Ctrl Pts',(17.5464540946258,16.9414388388218,-2.49462378750285));
#51075=CARTESIAN_POINT('Ctrl Pts',(17.4699743261962,16.9831320174928,-2.49893995025173));
#51076=CARTESIAN_POINT('Ctrl Pts',(17.3958663510844,17.0285705423451,-2.50325611300061));
#51077=CARTESIAN_POINT('Ctrl Pts',(17.3241724357532,17.0725289118542,-2.50743167718527));
#51078=CARTESIAN_POINT('Ctrl Pts',(17.2546985266629,17.1199920607128,-2.51160724136992));
#51079=CARTESIAN_POINT('Ctrl Pts',(17.1877934784099,17.1706947795508,-2.51578280555458));
#51080=CARTESIAN_POINT('Ctrl Pts',(17.1175092148074,17.2239583724966,-2.52016926758558));
#51081=CARTESIAN_POINT('Ctrl Pts',(17.0500605848372,17.2807970211557,-2.52455572961657));
#51082=CARTESIAN_POINT('Ctrl Pts',(16.9858097729217,17.3408580455089,-2.52894219164757));
#51083=CARTESIAN_POINT('Ctrl Pts',(16.9215589610061,17.4009190698621,-2.53332865367856));
#51084=CARTESIAN_POINT('Ctrl Pts',(16.8605063152544,17.4642019995291,-2.53771511570956));
#51085=CARTESIAN_POINT('Ctrl Pts',(16.802965079949,17.53031438468,-2.54210157774055));
#51086=CARTESIAN_POINT('Ctrl Pts',(16.7485317522924,17.5928559186595,-2.54625111891253));
#51087=CARTESIAN_POINT('Ctrl Pts',(16.6970294692197,17.6581717364498,-2.55040066008451));
#51088=CARTESIAN_POINT('Ctrl Pts',(16.6487573722079,17.7259534743858,-2.55455020125649));
#51089=CARTESIAN_POINT('Ctrl Pts',(16.600549374283,17.7936452069609,-2.55869423237573));
#51090=CARTESIAN_POINT('Ctrl Pts',(16.5555633203294,17.8637959851695,-2.56283826349497));
#51091=CARTESIAN_POINT('Ctrl Pts',(16.5140597201748,17.9360626862432,-2.56698229461421));
#51092=CARTESIAN_POINT('Ctrl Pts',(16.4725982721945,18.0082559913085,-2.57112211694382));
#51093=CARTESIAN_POINT('Ctrl Pts',(16.4346124893249,18.0825605501313,-2.57526193927342));
#51094=CARTESIAN_POINT('Ctrl Pts',(16.4003201033264,18.1586036203684,-2.57940176160303));
#51095=CARTESIAN_POINT('Ctrl Pts',(16.3660518421391,18.2345931940449,-2.58353867155343));
#51096=CARTESIAN_POINT('Ctrl Pts',(16.3354720095434,18.3123184246929,-2.58767558150382));
#51097=CARTESIAN_POINT('Ctrl Pts',(16.3087521158413,18.3913825890187,-2.59181249145422));
#51098=CARTESIAN_POINT('Ctrl Pts',(16.2820372325134,18.4704319276473,-2.59594862567298));
#51099=CARTESIAN_POINT('Ctrl Pts',(16.2591810094474,18.5508192612106,-2.60008475989173));
#51100=CARTESIAN_POINT('Ctrl Pts',(16.2403061251843,18.6321296702138,-2.60422089411049));
#51101=CARTESIAN_POINT('Ctrl Pts',(16.2214331728159,18.7134317568803,-2.6083566049849));
#51102=CARTESIAN_POINT('Ctrl Pts',(16.2065408484307,18.7956562735366,-2.61249231585931));
#51103=CARTESIAN_POINT('Ctrl Pts',(16.1957010120579,18.878376717874,-2.61662802673372));
#51104=CARTESIAN_POINT('Ctrl Pts',(16.1848552750843,18.9611421905962,-2.62076598885789));
#51105=CARTESIAN_POINT('Ctrl Pts',(16.1780664813585,19.0444036643639,-2.62490395098206));
#51106=CARTESIAN_POINT('Ctrl Pts',(16.175354661978,19.1277291514511,-2.62904191310623));
#51107=CARTESIAN_POINT('Ctrl Pts',(16.1744266413965,19.1562442389712,-2.63045797866132));
#51108=CARTESIAN_POINT('Ctrl Pts',(16.1739756253558,19.1847668138065,-2.63187404421641));
#51109=CARTESIAN_POINT('Ctrl Pts',(16.1740010149441,19.213279586128,-2.6332901097715));
#51110=CARTESIAN_POINT('Ctrl Pts',(16.1740010149447,19.2132795868243,-2.63329010980609));
#51111=CARTESIAN_POINT('Ctrl Pts',(16.1740928743929,19.3164386732002,-2.6384134288319));
#51112=CARTESIAN_POINT('Ctrl Pts',(16.1804238944875,19.4193213099348,-2.64353674785771));
#51113=CARTESIAN_POINT('Ctrl Pts',(16.1928719236876,19.5212710102101,-2.64866006688352));
#51114=CARTESIAN_POINT('Ctrl Pts',(16.2055250386105,19.6249003681759,-2.65386779441843));
#51115=CARTESIAN_POINT('Ctrl Pts',(16.2244983314989,19.7275658814857,-2.65907552195333));
#51116=CARTESIAN_POINT('Ctrl Pts',(16.2496149571641,19.8286009706384,-2.66428324948824));
#51117=CARTESIAN_POINT('Ctrl Pts',(16.2576437833531,19.8608980307853,-2.66594796113282));
#51118=CARTESIAN_POINT('Ctrl Pts',(16.2662999939973,19.8930286552691,-2.6676126727774));
#51119=CARTESIAN_POINT('Ctrl Pts',(16.2755767948953,19.9249715292663,-2.66927738442198));
#51120=CARTESIAN_POINT('Ctrl Pts',(16.2988961609903,20.0052672671023,-2.67346201883521));
#51121=CARTESIAN_POINT('Ctrl Pts',(16.3261969265522,20.084568763058,-2.67764665324844));
#51122=CARTESIAN_POINT('Ctrl Pts',(16.3573766633344,20.1624523191503,-2.68183128766167));
#51123=CARTESIAN_POINT('Ctrl Pts',(16.3885120196228,20.240225017646,-2.68600996576606));
#51124=CARTESIAN_POINT('Ctrl Pts',(16.4235152107072,20.3165833617541,-2.69018864387045));
#51125=CARTESIAN_POINT('Ctrl Pts',(16.4622338002162,20.391117932039,-2.69436732197484));
#51126=CARTESIAN_POINT('Ctrl Pts',(16.5016463923758,20.4669884804673,-2.6986208998552));
#51127=CARTESIAN_POINT('Ctrl Pts',(16.5449087556001,20.5409687666981,-2.70287447773556));
#51128=CARTESIAN_POINT('Ctrl Pts',(16.5918084260801,20.6126473381798,-2.70712805561591));
#51129=CARTESIAN_POINT('Ctrl Pts',(16.6377988552166,20.6829362811212,-2.71129916961482));
#51130=CARTESIAN_POINT('Ctrl Pts',(16.6872865541289,20.7510115566489,-2.71547028361373));
#51131=CARTESIAN_POINT('Ctrl Pts',(16.7400252973105,20.8165107863339,-2.71964139761264));
#51132=CARTESIAN_POINT('Ctrl Pts',(16.7927463434994,20.8819880371221,-2.72381111195412));
#51133=CARTESIAN_POINT('Ctrl Pts',(16.848715979104,20.9448906007935,-2.7279808262956));
#51134=CARTESIAN_POINT('Ctrl Pts',(16.907646512581,21.0048876606389,-2.73215054063707));
#51135=CARTESIAN_POINT('Ctrl Pts',(16.9665749490584,21.0648825855331,-2.73632010660234));
#51136=CARTESIAN_POINT('Ctrl Pts',(17.0284637509525,21.1219718845682,-2.74048967256761));
#51137=CARTESIAN_POINT('Ctrl Pts',(17.0929880053961,21.1758612250147,-2.74465923853288));
#51138=CARTESIAN_POINT('Ctrl Pts',(17.1597808523044,21.2316452475883,-2.74897540124709));
#51139=CARTESIAN_POINT('Ctrl Pts',(17.2293975200615,21.2839997657393,-2.7532915639613));
#51140=CARTESIAN_POINT('Ctrl Pts',(17.3014414464079,21.3326446428491,-2.75760772667551));
#51141=CARTESIAN_POINT('Ctrl Pts',(17.3711385501858,21.3797049187129,-2.76178329088849));
#51142=CARTESIAN_POINT('Ctrl Pts',(17.4431067778014,21.4232933214559,-2.76595885510147));
#51143=CARTESIAN_POINT('Ctrl Pts',(17.5169602827148,21.4632021060621,-2.77013441931445));
#51144=CARTESIAN_POINT('Ctrl Pts',(17.5945439513518,21.5051265878347,-2.77452088127928));
#51145=CARTESIAN_POINT('Ctrl Pts',(17.6742078257196,21.5429897170844,-2.77890734324411));
#51146=CARTESIAN_POINT('Ctrl Pts',(17.7554809190361,21.5766078305986,-2.78329380520893));
#51147=CARTESIAN_POINT('Ctrl Pts',(17.8367540123527,21.6102259441129,-2.78768026717376));
#51148=CARTESIAN_POINT('Ctrl Pts',(17.9196357523206,21.639598919772,-2.79206672913859));
#51149=CARTESIAN_POINT('Ctrl Pts',(18.0036392138267,21.6646041086574,-2.79645319110342));
#51150=CARTESIAN_POINT('Ctrl Pts',(18.0837805456624,21.6884596629898,-2.80063798179663));
#51151=CARTESIAN_POINT('Ctrl Pts',(18.1652410320985,21.7084290356245,-2.80482277248983));
#51152=CARTESIAN_POINT('Ctrl Pts',(18.2476089212223,21.7243689976773,-2.80900756318304));
#51153=CARTESIAN_POINT('Ctrl Pts',(18.329858738654,21.7402861103125,-2.81318635511479));
#51154=CARTESIAN_POINT('Ctrl Pts',(18.4130129271253,21.7521851992249,-2.81736514704654));
#51155=CARTESIAN_POINT('Ctrl Pts',(18.4966446832044,21.7599728232347,-2.82154393897828));
#51156=CARTESIAN_POINT('Ctrl Pts',(18.5801762046835,21.7677511135963,-2.82571772253095));
#51157=CARTESIAN_POINT('Ctrl Pts',(18.6641837002169,21.7714276931344,-2.82989150608361));
#51158=CARTESIAN_POINT('Ctrl Pts',(18.7482317172097,21.770960440754,-2.83406528963627));
#51159=CARTESIAN_POINT('Ctrl Pts',(18.8322246249339,21.7704934947452,-2.83823633648952));
#51160=CARTESIAN_POINT('Ctrl Pts',(18.9162575426888,21.7658881143946,-2.84240738334278));
#51161=CARTESIAN_POINT('Ctrl Pts',(18.9998925087996,21.7571541928493,-2.84657843019603));
#51162=CARTESIAN_POINT('Ctrl Pts',(19.0834977254746,21.7484233780099,-2.85074799338406));
#51163=CARTESIAN_POINT('Ctrl Pts',(19.1667048146448,21.7355669871508,-2.85491755657209));
#51164=CARTESIAN_POINT('Ctrl Pts',(19.2490798028149,21.7186468644393,-2.85908711976013));
#51165=CARTESIAN_POINT('Ctrl Pts',(19.3314501999326,21.7017276847466,-2.86325645056351));
#51166=CARTESIAN_POINT('Ctrl Pts',(19.4129881380694,21.6807453176226,-2.8674257813669));
#51167=CARTESIAN_POINT('Ctrl Pts',(19.4932700684876,21.6558126642135,-2.87159511217028));
#51168=CARTESIAN_POINT('Ctrl Pts',(19.5736163334739,21.6308600308229,-2.87576778410031));
#51169=CARTESIAN_POINT('Ctrl Pts',(19.6527041405867,21.6019509257347,-2.87994045603033));
#51170=CARTESIAN_POINT('Ctrl Pts',(19.7301259599786,21.5692478817666,-2.88411312796035));
#51171=CARTESIAN_POINT('Ctrl Pts',(19.8075810658885,21.5365307775443,-2.88828759387715));
#51172=CARTESIAN_POINT('Ctrl Pts',(19.8833683419578,21.5000166836297,-2.89246205979394));
#51173=CARTESIAN_POINT('Ctrl Pts',(19.9571031322698,21.4599150112514,-2.89663652571074));
#51174=CARTESIAN_POINT('Ctrl Pts',(20.0309449059695,21.4197551544971,-2.9008170484496));
#51175=CARTESIAN_POINT('Ctrl Pts',(20.1027278532631,21.3759975629064,-2.90499757118846));
#51176=CARTESIAN_POINT('Ctrl Pts',(20.1720950490314,21.3288958024302,-2.90917809392733));
#51177=CARTESIAN_POINT('Ctrl Pts',(20.2134569395969,21.3008102233509,-2.91167083306888));
#51178=CARTESIAN_POINT('Ctrl Pts',(20.2539605167435,21.2715364569413,-2.91416357221043));
#51179=CARTESIAN_POINT('Ctrl Pts',(20.2935358855687,21.2411349269503,-2.91665631135199));
#51180=CARTESIAN_POINT('',(16.1740009418753,19.2088040034395,-2.56670989022851));
#51181=CARTESIAN_POINT('Ctrl Pts',(16.17268506744,19.2088155460777,-2.56671052147119));
#51182=CARTESIAN_POINT('Ctrl Pts',(16.1790130470455,19.904586810716,-2.60137099441749));
#51183=CARTESIAN_POINT('Ctrl Pts',(16.8320815026504,21.4617759084344,-2.67842340292429));
#51184=CARTESIAN_POINT('Ctrl Pts',(18.916759365406,22.004542103009,-2.77291032493482));
#51185=CARTESIAN_POINT('Ctrl Pts',(20.0133687968266,21.4537986792987,-2.83273677399906));
#51186=CARTESIAN_POINT('Ctrl Pts',(20.2912843055177,21.2382340775644,-2.85017128750281));
#51187=CARTESIAN_POINT('Ctrl Pts',(20.2935358855687,21.2411349269503,-2.05017637612677));
#51188=CARTESIAN_POINT('Ctrl Pts',(20.359994771256,21.1900816615893,-2.05435390919074));
#51189=CARTESIAN_POINT('Ctrl Pts',(20.4240373077701,21.1356899351298,-2.05853144225471));
#51190=CARTESIAN_POINT('Ctrl Pts',(20.4853117216981,21.0782191230391,-2.06270897531868));
#51191=CARTESIAN_POINT('Ctrl Pts',(20.5465213891913,21.0208090382561,-2.06688209413607));
#51192=CARTESIAN_POINT('Ctrl Pts',(20.6049684136104,20.9603266476494,-2.07105521295346));
#51193=CARTESIAN_POINT('Ctrl Pts',(20.6603338871675,20.8970716933601,-2.07522833177086));
#51194=CARTESIAN_POINT('Ctrl Pts',(20.7156675768893,20.8338530520456,-2.07939905491252));
#51195=CARTESIAN_POINT('Ctrl Pts',(20.7679229256929,20.7678653524743,-2.08356977805419));
#51196=CARTESIAN_POINT('Ctrl Pts',(20.816818521466,20.6994444922933,-2.08774050119586));
#51197=CARTESIAN_POINT('Ctrl Pts',(20.8657007153038,20.6310423857838,-2.09191008117196));
#51198=CARTESIAN_POINT('Ctrl Pts',(20.9112247179256,20.5602088174111,-2.09607966114805));
#51199=CARTESIAN_POINT('Ctrl Pts',(20.9531508438531,20.4873109073522,-2.10024924112415));
#51200=CARTESIAN_POINT('Ctrl Pts',(20.9950780549202,20.4144111105363,-2.10441892901808));
#51201=CARTESIAN_POINT('Ctrl Pts',(21.0334069761503,20.3394472653802,-2.10858861691201));
#51202=CARTESIAN_POINT('Ctrl Pts',(21.0679432142698,20.2628122800976,-2.11275830480594));
#51203=CARTESIAN_POINT('Ctrl Pts',(21.1025145449794,20.1860994252995,-2.11693222955821));
#51204=CARTESIAN_POINT('Ctrl Pts',(21.1332853054147,20.1077124589645,-2.12110615431048));
#51205=CARTESIAN_POINT('Ctrl Pts',(21.1601089494097,20.0280650926297,-2.12528007906274));
#51206=CARTESIAN_POINT('Ctrl Pts',(21.1869458971437,19.9483782235423,-2.129456073959));
#51207=CARTESIAN_POINT('Ctrl Pts',(21.2098317036757,19.8674301524326,-2.13363206885525));
#51208=CARTESIAN_POINT('Ctrl Pts',(21.2286701984997,19.7856482408549,-2.13780806375151));
#51209=CARTESIAN_POINT('Ctrl Pts',(21.2475424627081,19.7037197291988,-2.14199154442509));
#51210=CARTESIAN_POINT('Ctrl Pts',(21.2623528375578,19.6209548443099,-2.14617502509867));
#51211=CARTESIAN_POINT('Ctrl Pts',(21.273056640058,19.537789501939,-2.15035850577225));
#51212=CARTESIAN_POINT('Ctrl Pts',(21.2829756092266,19.4607220796968,-2.15423524170963));
#51213=CARTESIAN_POINT('Ctrl Pts',(21.2893686863835,19.3833111209002,-2.158111977647));
#51214=CARTESIAN_POINT('Ctrl Pts',(21.292240293453,19.3059031135093,-2.16198871358438));
#51215=CARTESIAN_POINT('Ctrl Pts',(21.2953399702058,19.2223471829115,-2.16617334886756));
#51216=CARTESIAN_POINT('Ctrl Pts',(21.2943475192288,19.1384837390471,-2.17035798415075));
#51217=CARTESIAN_POINT('Ctrl Pts',(21.2892270081185,19.0547472016827,-2.17454261943394));
#51218=CARTESIAN_POINT('Ctrl Pts',(21.2841137854076,18.9711298526819,-2.17872129841839));
#51219=CARTESIAN_POINT('Ctrl Pts',(21.2748842015326,18.88763950663,-2.18289997740284));
#51220=CARTESIAN_POINT('Ctrl Pts',(21.2615542857283,18.8047127460814,-2.18707865638728));
#51221=CARTESIAN_POINT('Ctrl Pts',(21.2479854444013,18.7202996055814,-2.19133223404889));
#51222=CARTESIAN_POINT('Ctrl Pts',(21.2301678127982,18.6364709353496,-2.19558581171049));
#51223=CARTESIAN_POINT('Ctrl Pts',(21.2081737664701,18.5536841145149,-2.1998393893721));
#51224=CARTESIAN_POINT('Ctrl Pts',(21.1866061117593,18.4725022555819,-2.20401050426942));
#51225=CARTESIAN_POINT('Ctrl Pts',(21.1610226544981,18.3923226756034,-2.20818161916673));
#51226=CARTESIAN_POINT('Ctrl Pts',(21.1315432452061,18.3135667783247,-2.21235273406405));
#51227=CARTESIAN_POINT('Ctrl Pts',(21.1020737279769,18.2348373082472,-2.21652244930882));
#51228=CARTESIAN_POINT('Ctrl Pts',(21.0687110162085,18.1575310025734,-2.22069216455359));
#51229=CARTESIAN_POINT('Ctrl Pts',(21.0316242450291,18.0820523357327,-2.22486187979835));
#51230=CARTESIAN_POINT('Ctrl Pts',(20.9945387935218,18.0065763546772,-2.2290314466706));
#51231=CARTESIAN_POINT('Ctrl Pts',(20.9537297497136,17.9329282956594,-2.23320101354286));
#51232=CARTESIAN_POINT('Ctrl Pts',(20.9094130508257,17.861489696854,-2.23737058041511));
#51233=CARTESIAN_POINT('Ctrl Pts',(20.8635382532167,17.7875394400905,-2.24168674206933));
#51234=CARTESIAN_POINT('Ctrl Pts',(20.8139048345105,17.7159573495152,-2.24600290372356));
#51235=CARTESIAN_POINT('Ctrl Pts',(20.7608012117929,17.6471340057809,-2.25031906537778));
#51236=CARTESIAN_POINT('Ctrl Pts',(20.7094274096687,17.5805525436961,-2.25449463049769));
#51237=CARTESIAN_POINT('Ctrl Pts',(20.6548063540235,17.5165531862989,-2.25867019561761));
#51238=CARTESIAN_POINT('Ctrl Pts',(20.5972390426215,17.4554544238184,-2.26284576073752));
#51239=CARTESIAN_POINT('Ctrl Pts',(20.5367641854478,17.3912697529606,-2.2672322206589));
#51240=CARTESIAN_POINT('Ctrl Pts',(20.4730380462776,17.3302867949802,-2.27161868058029));
#51241=CARTESIAN_POINT('Ctrl Pts',(20.4064500166287,17.27282793801,-2.27600514050167));
#51242=CARTESIAN_POINT('Ctrl Pts',(20.3398619869799,17.2153690810398,-2.28039160042305));
#51243=CARTESIAN_POINT('Ctrl Pts',(20.2704125717623,17.161434620885,-2.28477806034443));
#51244=CARTESIAN_POINT('Ctrl Pts',(20.1985254700647,17.1112940330771,-2.28916452026581));
#51245=CARTESIAN_POINT('Ctrl Pts',(20.1299459675149,17.0634604650486,-2.29334915467531));
#51246=CARTESIAN_POINT('Ctrl Pts',(20.0588929044646,17.0189012759396,-2.2975337890848));
#51247=CARTESIAN_POINT('Ctrl Pts',(19.9857121094414,16.9778818224111,-2.3017184234943));
#51248=CARTESIAN_POINT('Ctrl Pts',(19.9126354781723,16.9369207549698,-2.30589710159751));
#51249=CARTESIAN_POINT('Ctrl Pts',(19.8374375284665,16.8994896383239,-2.31007577970071));
#51250=CARTESIAN_POINT('Ctrl Pts',(19.7604940332793,16.8658113083076,-2.31425445780392));
#51251=CARTESIAN_POINT('Ctrl Pts',(19.6821713816824,16.8315293186239,-2.31850803568489));
#51252=CARTESIAN_POINT('Ctrl Pts',(19.6020403867561,16.8011362520523,-2.32276161356587));
#51253=CARTESIAN_POINT('Ctrl Pts',(19.5205248076185,16.7748188230346,-2.32701519144684));
#51254=CARTESIAN_POINT('Ctrl Pts',(19.4405895664632,16.7490116085441,-2.33118630545089));
#51255=CARTESIAN_POINT('Ctrl Pts',(19.3593234056723,16.7271235613564,-2.33535741945493));
#51256=CARTESIAN_POINT('Ctrl Pts',(19.2771455317487,16.7092820040337,-2.33952853345898));
#51257=CARTESIAN_POINT('Ctrl Pts',(19.1949952333547,16.6914464336072,-2.34369824780796));
#51258=CARTESIAN_POINT('Ctrl Pts',(19.1119342786025,16.6776547538833,-2.34786796215693));
#51259=CARTESIAN_POINT('Ctrl Pts',(19.0283943159519,16.6679836833525,-2.3520376765059));
#51260=CARTESIAN_POINT('Ctrl Pts',(18.9448573259619,16.6583129569542,-2.35620724248102));
#51261=CARTESIAN_POINT('Ctrl Pts',(18.8608418190422,16.6527626002741,-2.36037680845614));
#51262=CARTESIAN_POINT('Ctrl Pts',(18.7767854909837,16.6513575636896,-2.36454637443126));
#51263=CARTESIAN_POINT('Ctrl Pts',(18.6897738473637,16.6499031277727,-2.36886253714093));
#51264=CARTESIAN_POINT('Ctrl Pts',(18.602718986005,16.6528909431625,-2.3731786998506));
#51265=CARTESIAN_POINT('Ctrl Pts',(18.516105438621,16.6602899106089,-2.37749486256026));
#51266=CARTESIAN_POINT('Ctrl Pts',(18.4323133171228,16.6674478575809,-2.38167042678893));
#51267=CARTESIAN_POINT('Ctrl Pts',(18.3489346599913,16.6787338735485,-2.3858459910176));
#51268=CARTESIAN_POINT('Ctrl Pts',(18.2664001913304,16.694067259752,-2.39002155524626));
#51269=CARTESIAN_POINT('Ctrl Pts',(18.1796971048655,16.7101750984693,-2.39440801719643));
#51270=CARTESIAN_POINT('Ctrl Pts',(18.0939262957202,16.7307497815375,-2.39879447914659));
#51271=CARTESIAN_POINT('Ctrl Pts',(18.0095696123178,16.7556383945735,-2.40318094109676));
#51272=CARTESIAN_POINT('Ctrl Pts',(17.9252129289154,16.7805270076095,-2.40756740304692));
#51273=CARTESIAN_POINT('Ctrl Pts',(17.8422708932813,16.8097292861762,-2.41195386499709));
#51274=CARTESIAN_POINT('Ctrl Pts',(17.7611994326656,16.8430348279179,-2.41634032694725));
#51275=CARTESIAN_POINT('Ctrl Pts',(17.6838581936306,16.8748079308751,-2.42052496109137));
#51276=CARTESIAN_POINT('Ctrl Pts',(17.6079312972171,16.9104332654877,-2.42470959523549));
#51277=CARTESIAN_POINT('Ctrl Pts',(17.5338290567806,16.9497636773101,-2.4288942293796));
#51278=CARTESIAN_POINT('Ctrl Pts',(17.4598322917951,16.9890381071151,-2.43307290721024));
#51279=CARTESIAN_POINT('Ctrl Pts',(17.3876554268513,17.0320069250301,-2.43725158504088));
#51280=CARTESIAN_POINT('Ctrl Pts',(17.3176892303787,17.0784747823637,-2.44143026287152));
#51281=CARTESIAN_POINT('Ctrl Pts',(17.2464689347497,17.1257755462096,-2.44568384081973));
#51282=CARTESIAN_POINT('Ctrl Pts',(17.1775397858983,17.1767018411992,-2.44993741876795));
#51283=CARTESIAN_POINT('Ctrl Pts',(17.1112881539821,17.2309984179822,-2.45419099671616));
#51284=CARTESIAN_POINT('Ctrl Pts',(17.046320944273,17.2842423455401,-2.45836211043189));
#51285=CARTESIAN_POINT('Ctrl Pts',(16.9839287319629,17.3407267365349,-2.46253322414762));
#51286=CARTESIAN_POINT('Ctrl Pts',(16.9244454837024,17.4001680220001,-2.46670433786335));
#51287=CARTESIAN_POINT('Ctrl Pts',(16.864982195661,17.4595893613273,-2.47087405191874));
#51288=CARTESIAN_POINT('Ctrl Pts',(16.80842625819,17.5219652996602,-2.47504376597413));
#51289=CARTESIAN_POINT('Ctrl Pts',(16.7550758225251,17.5869744152861,-2.47921348002952));
#51290=CARTESIAN_POINT('Ctrl Pts',(16.7017272853287,17.6519812175709,-2.48338304570617));
#51291=CARTESIAN_POINT('Ctrl Pts',(16.6515843143223,17.7196206546924,-2.48755261138281));
#51292=CARTESIAN_POINT('Ctrl Pts',(16.6049048052609,17.789538198987,-2.49172217705945));
#51293=CARTESIAN_POINT('Ctrl Pts',(16.5565840956936,17.8619139677013,-2.49603834010689));
#51294=CARTESIAN_POINT('Ctrl Pts',(16.5119752240704,17.9367305827085,-2.50035450315433));
#51295=CARTESIAN_POINT('Ctrl Pts',(16.4713143087829,18.0135637959534,-2.50467066620176));
#51296=CARTESIAN_POINT('Ctrl Pts',(16.4319779238963,18.087894165226,-2.50884623012272));
#51297=CARTESIAN_POINT('Ctrl Pts',(16.3963363916594,18.1641113217507,-2.51302179404367));
#51298=CARTESIAN_POINT('Ctrl Pts',(16.3645549999772,18.241809414064,-2.51719735796462));
#51299=CARTESIAN_POINT('Ctrl Pts',(16.331168399037,18.3234318687324,-2.5215838205753));
#51300=CARTESIAN_POINT('Ctrl Pts',(16.3020423326827,18.4066882445185,-2.52597028318598));
#51301=CARTESIAN_POINT('Ctrl Pts',(16.2773090396161,18.491090613224,-2.53035674579666));
#51302=CARTESIAN_POINT('Ctrl Pts',(16.2525757465496,18.5754929819294,-2.53474320840733));
#51303=CARTESIAN_POINT('Ctrl Pts',(16.2322352869838,18.6610407614778,-2.53912967101801));
#51304=CARTESIAN_POINT('Ctrl Pts',(16.2163575306379,18.7472367021162,-2.54351613362869));
#51305=CARTESIAN_POINT('Ctrl Pts',(16.1935441105101,18.8710844400618,-2.54981867488401));
#51306=CARTESIAN_POINT('Ctrl Pts',(16.179864182312,18.9966631544576,-2.55612121613934));
#51307=CARTESIAN_POINT('Ctrl Pts',(16.1755170133968,19.1228818562274,-2.56242375739466));
#51308=CARTESIAN_POINT('Ctrl Pts',(16.1745315620438,19.1514941307573,-2.56385246833928));
#51309=CARTESIAN_POINT('Ctrl Pts',(16.1740255308992,19.180139168944,-2.56528117928389));
#51310=CARTESIAN_POINT('Ctrl Pts',(16.1740009418753,19.2088040034395,-2.56670989022851));
#51311=CARTESIAN_POINT('Origin',(18.734,19.211,1.76670989022852));
#51312=CARTESIAN_POINT('',(20.2935358855687,21.2411349269503,-1.25003886315632));
#51313=CARTESIAN_POINT('',(20.2916962525237,21.2387762312159,-1.31677679826697));
#51314=CARTESIAN_POINT('',(20.2935358855687,21.2411349269503,1.76670989022852));
#51315=CARTESIAN_POINT('',(16.1742339456424,19.2099923322427,-1.83329006740172));
#51316=CARTESIAN_POINT('Ctrl Pts',(20.2916962525238,21.2387762312158,-1.31677679826698));
#51317=CARTESIAN_POINT('Ctrl Pts',(20.71974029023,20.9053211442369,-1.34369097138053));
#51318=CARTESIAN_POINT('Ctrl Pts',(21.5659317303477,19.7058144822129,-1.41299708005456));
#51319=CARTESIAN_POINT('Ctrl Pts',(21.0139855967169,17.219779463867,-1.52469512428907));
#51320=CARTESIAN_POINT('Ctrl Pts',(18.2938122975693,16.2160838163956,-1.65187093097051));
#51321=CARTESIAN_POINT('Ctrl Pts',(16.4202753011031,17.6266608733541,-1.75473569408333));
#51322=CARTESIAN_POINT('Ctrl Pts',(16.1765569575323,18.8451666316293,-1.81520852163568));
#51323=CARTESIAN_POINT('Ctrl Pts',(16.1778407186761,19.2099805598359,-1.83328941362754));
#51324=CARTESIAN_POINT('Ctrl Pts',(16.174000198019,19.2099930951884,-1.8332901097715));
#51325=CARTESIAN_POINT('Ctrl Pts',(16.1739663681253,19.2960037291259,-1.83754657623673));
#51326=CARTESIAN_POINT('Ctrl Pts',(16.1782715498352,19.3819895204514,-1.84180304270196));
#51327=CARTESIAN_POINT('Ctrl Pts',(16.1868819594924,19.4674950052547,-1.84605950916719));
#51328=CARTESIAN_POINT('Ctrl Pts',(16.1954973714593,19.5530501653856,-1.85031844847222));
#51329=CARTESIAN_POINT('Ctrl Pts',(16.2084229438551,19.6381240334814,-1.85457738777724));
#51330=CARTESIAN_POINT('Ctrl Pts',(16.2255732751461,19.7222683894382,-1.85883632708227));
#51331=CARTESIAN_POINT('Ctrl Pts',(16.2427520342423,19.8065522202146,-1.86310232586009));
#51332=CARTESIAN_POINT('Ctrl Pts',(16.2641694501953,19.8899030371078,-1.86736832463791));
#51333=CARTESIAN_POINT('Ctrl Pts',(16.2896893999656,19.9718848076808,-1.87163432341573));
#51334=CARTESIAN_POINT('Ctrl Pts',(16.3152317962993,20.0539386868993,-1.87590407443496));
#51335=CARTESIAN_POINT('Ctrl Pts',(16.3448837660451,20.1346207148683,-1.88017382545418));
#51336=CARTESIAN_POINT('Ctrl Pts',(16.378460747601,20.2135142544661,-1.8844435764734));
#51337=CARTESIAN_POINT('Ctrl Pts',(16.4121081360956,20.2925732244374,-1.88872228065292));
#51338=CARTESIAN_POINT('Ctrl Pts',(16.4496967908718,20.3698358236637,-1.89300098483243));
#51339=CARTESIAN_POINT('Ctrl Pts',(16.4909957509127,20.4449092100217,-1.89727968901195));
#51340=CARTESIAN_POINT('Ctrl Pts',(16.5197685295451,20.4972124623244,-1.90026064078576));
#51341=CARTESIAN_POINT('Ctrl Pts',(16.5503412786202,20.5484536572702,-1.90324159255957));
#51342=CARTESIAN_POINT('Ctrl Pts',(16.5826239200438,20.5985089054101,-1.90622254433338));
#51343=CARTESIAN_POINT('Ctrl Pts',(16.6279420233601,20.668776046099,-1.9104071796206));
#51344=CARTESIAN_POINT('Ctrl Pts',(16.6767906254528,20.7369513808156,-1.91459181490782));
#51345=CARTESIAN_POINT('Ctrl Pts',(16.728950354716,20.8026582296292,-1.91877645019504));
#51346=CARTESIAN_POINT('Ctrl Pts',(16.7810358412062,20.8682715530599,-1.92295512918357));
#51347=CARTESIAN_POINT('Ctrl Pts',(16.8364228098493,20.9314230124315,-1.9271338081721));
#51348=CARTESIAN_POINT('Ctrl Pts',(16.8948480567163,20.9917639174006,-1.93131248716063));
#51349=CARTESIAN_POINT('Ctrl Pts',(16.9543205181259,21.0531863731818,-1.93556606482122));
#51350=CARTESIAN_POINT('Ctrl Pts',(17.016940988373,21.1116961215207,-1.93981964248181));
#51351=CARTESIAN_POINT('Ctrl Pts',(17.0823881640281,21.1669596987866,-1.9440732201424));
#51352=CARTESIAN_POINT('Ctrl Pts',(17.1465665360758,21.2211518986326,-1.94824433504389));
#51353=CARTESIAN_POINT('Ctrl Pts',(17.2134626230229,21.2722223587369,-1.95241544994537));
#51354=CARTESIAN_POINT('Ctrl Pts',(17.2827368115688,21.3198942974707,-1.95658656484686));
#51355=CARTESIAN_POINT('Ctrl Pts',(17.3519877545808,21.3675502394864,-1.96075628009582));
#51356=CARTESIAN_POINT('Ctrl Pts',(17.4236148357134,21.4118096644133,-1.96492599534479));
#51357=CARTESIAN_POINT('Ctrl Pts',(17.497247739258,21.4524378968754,-1.96909571059375));
#51358=CARTESIAN_POINT('Ctrl Pts',(17.5708780226959,21.4930646836483,-1.97326527747021));
#51359=CARTESIAN_POINT('Ctrl Pts',(17.6465135834374,21.5300603133606,-1.97743484434667));
#51360=CARTESIAN_POINT('Ctrl Pts',(17.7237588789492,21.5632357189146,-1.98160441122312));
#51361=CARTESIAN_POINT('Ctrl Pts',(17.8037199856914,21.5975775144525,-1.98592057287243));
#51362=CARTESIAN_POINT('Ctrl Pts',(17.8854056436194,21.6278252451695,-1.99023673452174));
#51363=CARTESIAN_POINT('Ctrl Pts',(17.9683557183338,21.6538239465733,-1.99455289617105));
#51364=CARTESIAN_POINT('Ctrl Pts',(18.0486037412681,21.6789757549796,-1.99872846129518));
#51365=CARTESIAN_POINT('Ctrl Pts',(18.1300346026431,21.7001510305579,-2.00290402641931));
#51366=CARTESIAN_POINT('Ctrl Pts',(18.2122191472962,21.7172611080555,-2.00707959154345));
#51367=CARTESIAN_POINT('Ctrl Pts',(18.2985545772993,21.7352353622706,-2.01146605145534));
#51368=CARTESIAN_POINT('Ctrl Pts',(18.3857212504014,21.7487228766122,-2.01585251136724));
#51369=CARTESIAN_POINT('Ctrl Pts',(18.4732153214809,21.7576824206111,-2.02023897127913));
#51370=CARTESIAN_POINT('Ctrl Pts',(18.5607093925604,21.7666419646101,-2.02462543119103));
#51371=CARTESIAN_POINT('Ctrl Pts',(18.6485302783063,21.7710735849926,-2.02901189110292));
#51372=CARTESIAN_POINT('Ctrl Pts',(18.7361763184418,21.7709990749291,-2.03339835101482));
#51373=CARTESIAN_POINT('Ctrl Pts',(18.8197745701698,21.7709280059906,-2.03758222948032));
#51374=CARTESIAN_POINT('Ctrl Pts',(18.903524881571,21.7667575762853,-2.04176610794582));
#51375=CARTESIAN_POINT('Ctrl Pts',(18.9869920193077,21.7584683586193,-2.04594998641132));
#51376=CARTESIAN_POINT('Ctrl Pts',(19.0703479391422,21.7501901861314,-2.05012828996198));
#51377=CARTESIAN_POINT('Ctrl Pts',(19.1534209809432,21.7378041671254,-2.05430659351263));
#51378=CARTESIAN_POINT('Ctrl Pts',(19.2357756009639,21.7213428543283,-2.05848489706328));
#51379=CARTESIAN_POINT('Ctrl Pts',(19.3180452017791,21.7048985354502,-2.06265888712128));
#51380=CARTESIAN_POINT('Ctrl Pts',(19.3995974052585,21.6843873684876,-2.06683287717928));
#51381=CARTESIAN_POINT('Ctrl Pts',(19.4800028447563,21.659893577846,-2.07100686723728));
#51382=CARTESIAN_POINT('Ctrl Pts',(19.5603542148008,21.6354162583024,-2.07517805045333));
#51383=CARTESIAN_POINT('Ctrl Pts',(19.6395599135012,21.6069617675492,-2.07934923366938));
#51384=CARTESIAN_POINT('Ctrl Pts',(19.7172030732739,21.574664890949,-2.08352041688543));
#51385=CARTESIAN_POINT('Ctrl Pts',(19.7948145897919,21.5423811768513,-2.08768990014732));
#51386=CARTESIAN_POINT('Ctrl Pts',(19.8708644093505,21.5062583672899,-2.0918593834092));
#51387=CARTESIAN_POINT('Ctrl Pts',(19.9449544117907,21.4664798630368,-2.09602886667109));
#51388=CARTESIAN_POINT('Ctrl Pts',(20.0190582144985,21.4266939494979,-2.10019912655578));
#51389=CARTESIAN_POINT('Ctrl Pts',(20.0912010629143,21.3832511941884,-2.10436938644046));
#51390=CARTESIAN_POINT('Ctrl Pts',(20.1610091624564,21.3363811070642,-2.10853964632514));
#51391=CARTESIAN_POINT('Ctrl Pts',(20.206193956802,21.306043434766,-2.11123893675839));
#51392=CARTESIAN_POINT('Ctrl Pts',(20.2504011005482,21.2742707763279,-2.11393822719164));
#51393=CARTESIAN_POINT('Ctrl Pts',(20.2935358855687,21.2411349269503,-2.11663751762489));
#51394=CARTESIAN_POINT('',(16.1740004726294,19.2125555906437,-1.76670989019937));
#51395=CARTESIAN_POINT('Ctrl Pts',(16.1740004726297,19.2125555912267,-1.7667098902285));
#51396=CARTESIAN_POINT('Ctrl Pts',(16.1740562220857,19.3043011464569,-1.77129369133236));
#51397=CARTESIAN_POINT('Ctrl Pts',(16.1790436176611,19.3958958077681,-1.77587749243622));
#51398=CARTESIAN_POINT('Ctrl Pts',(16.188916332748,19.4869513121681,-1.78046129354008));
#51399=CARTESIAN_POINT('Ctrl Pts',(16.1979293239672,19.5700776309547,-1.78464593360467));
#51400=CARTESIAN_POINT('Ctrl Pts',(16.2110359189468,19.6529166093026,-1.78883057366926));
#51401=CARTESIAN_POINT('Ctrl Pts',(16.2282088654964,19.7350331957452,-1.79301521373385));
#51402=CARTESIAN_POINT('Ctrl Pts',(16.2453573687607,19.8170329007231,-1.79719389754915));
#51403=CARTESIAN_POINT('Ctrl Pts',(16.2665606336754,19.898311809733,-1.80137258136445));
#51404=CARTESIAN_POINT('Ctrl Pts',(16.2917396796525,19.9784402437038,-1.80555126517975));
#51405=CARTESIAN_POINT('Ctrl Pts',(16.3173699981905,20.0600047830626,-1.80980484163982));
#51406=CARTESIAN_POINT('Ctrl Pts',(16.3471199654275,20.1403767219199,-1.8140584180999));
#51407=CARTESIAN_POINT('Ctrl Pts',(16.3808518403883,20.2191139513548,-1.81831199455997));
#51408=CARTESIAN_POINT('Ctrl Pts',(16.4139298144973,20.2963248398595,-1.82248311437409));
#51409=CARTESIAN_POINT('Ctrl Pts',(16.450836503808,20.3719633895875,-1.82665423418821));
#51410=CARTESIAN_POINT('Ctrl Pts',(16.4913923918018,20.4456299508969,-1.83082535400233));
#51411=CARTESIAN_POINT('Ctrl Pts',(16.5319346711508,20.5192717931798,-1.8349950741852));
#51412=CARTESIAN_POINT('Ctrl Pts',(16.5761234956298,20.5909425585429,-1.83916479436806));
#51413=CARTESIAN_POINT('Ctrl Pts',(16.6237330294819,20.6602664741656,-1.84333451455093));
#51414=CARTESIAN_POINT('Ctrl Pts',(16.671340869397,20.7295879232582,-1.84750408637604));
#51415=CARTESIAN_POINT('Ctrl Pts',(16.7223689155627,20.7965623098985,-1.85167365820116));
#51416=CARTESIAN_POINT('Ctrl Pts',(16.7765483378666,20.8608433229889,-1.85584323002627));
#51417=CARTESIAN_POINT('Ctrl Pts',(16.8326324731959,20.9273841771355,-1.86015938587588));
#51418=CARTESIAN_POINT('Ctrl Pts',(16.8920933523659,20.9910383498724,-1.86447554172548));
#51419=CARTESIAN_POINT('Ctrl Pts',(16.9545891221584,21.0514610639237,-1.86879169757509));
#51420=CARTESIAN_POINT('Ctrl Pts',(17.0150492802823,21.1099156898598,-1.872967267634));
#51421=CARTESIAN_POINT('Ctrl Pts',(17.0783492738879,21.1653458606137,-1.87714283769291));
#51422=CARTESIAN_POINT('Ctrl Pts',(17.1441452212348,21.2174799481773,-1.88131840775181));
#51423=CARTESIAN_POINT('Ctrl Pts',(17.2132640592835,21.2722469619589,-1.88570485649677));
#51424=CARTESIAN_POINT('Ctrl Pts',(17.2851371185139,21.323375865423,-1.89009130524172));
#51425=CARTESIAN_POINT('Ctrl Pts',(17.3593324933327,21.3706039558477,-1.89447775398667));
#51426=CARTESIAN_POINT('Ctrl Pts',(17.4335278681516,21.4178320462725,-1.89886420273162));
#51427=CARTESIAN_POINT('Ctrl Pts',(17.5100450161993,21.4611591039616,-1.90325065147657));
#51428=CARTESIAN_POINT('Ctrl Pts',(17.5884257348941,21.5003797420103,-1.90763710022152));
#51429=CARTESIAN_POINT('Ctrl Pts',(17.6632002791351,21.5377958997562,-1.91182173531038));
#51430=CARTESIAN_POINT('Ctrl Pts',(17.7399490034729,21.5716144630813,-1.91600637039924));
#51431=CARTESIAN_POINT('Ctrl Pts',(17.818291348554,21.6016228614457,-1.9201910054881));
#51432=CARTESIAN_POINT('Ctrl Pts',(17.8965221835546,21.6315885467804,-1.92436968429629));
#51433=CARTESIAN_POINT('Ctrl Pts',(17.9763417077984,21.6577546763325,-1.92854836310447));
#51434=CARTESIAN_POINT('Ctrl Pts',(18.0573458795764,21.679955082887,-1.93272704191266));
#51435=CARTESIAN_POINT('Ctrl Pts',(18.1398019751846,21.7025534109142,-1.93698061962059));
#51436=CARTESIAN_POINT('Ctrl Pts',(18.22348517397,21.7210422324029,-1.94123419732852));
#51437=CARTESIAN_POINT('Ctrl Pts',(18.3079491747639,21.7352980597219,-1.94548777503645));
#51438=CARTESIAN_POINT('Ctrl Pts',(18.3907756952125,21.7492775132387,-1.94965888980362));
#51439=CARTESIAN_POINT('Ctrl Pts',(18.4743525389348,21.759186555656,-1.95383000457078));
#51440=CARTESIAN_POINT('Ctrl Pts',(18.5582464958671,21.7649598089604,-1.95800111933795));
#51441=CARTESIAN_POINT('Ctrl Pts',(18.6421123018319,21.7707311250256,-1.96217083447015));
#51442=CARTESIAN_POINT('Ctrl Pts',(18.7262945511122,21.772369376577,-1.96634054960234));
#51443=CARTESIAN_POINT('Ctrl Pts',(18.8103550385056,21.769861056817,-1.97051026473454));
#51444=CARTESIAN_POINT('Ctrl Pts',(18.8944125351025,21.7673528263009,-1.97467983151203));
#51445=CARTESIAN_POINT('Ctrl Pts',(18.9783478186234,21.7606983323763,-1.97884939828952));
#51446=CARTESIAN_POINT('Ctrl Pts',(19.0617241844592,21.7499361667676,-1.983018965067));
#51447=CARTESIAN_POINT('Ctrl Pts',(19.1480319248283,21.7387956212922,-1.98733512688666));
#51448=CARTESIAN_POINT('Ctrl Pts',(19.2337401905612,21.7232532494629,-1.99165128870633));
#51449=CARTESIAN_POINT('Ctrl Pts',(19.3183740371403,21.7034098749436,-1.99596745052599));
#51450=CARTESIAN_POINT('Ctrl Pts',(19.4002509797481,21.6842128881312,-2.00014301559692));
#51451=CARTESIAN_POINT('Ctrl Pts',(19.481121986091,21.6609909777928,-2.00431858066785));
#51452=CARTESIAN_POINT('Ctrl Pts',(19.5605725242401,21.6338862668667,-2.00849414573879));
#51453=CARTESIAN_POINT('Ctrl Pts',(19.6440358680186,21.6054125792273,-2.01288060593281));
#51454=CARTESIAN_POINT('Ctrl Pts',(19.725930936615,21.572653764432,-2.01726706612684));
#51455=CARTESIAN_POINT('Ctrl Pts',(19.8058030522818,21.5358307932233,-2.02165352632086));
#51456=CARTESIAN_POINT('Ctrl Pts',(19.8856751679486,21.4990078220147,-2.02603998651489));
#51457=CARTESIAN_POINT('Ctrl Pts',(19.9635238523773,21.4581210315221,-2.03042644670891));
#51458=CARTESIAN_POINT('Ctrl Pts',(20.0389283879064,21.4134445287989,-2.03481290690294));
#51459=CARTESIAN_POINT('Ctrl Pts',(20.1108650768746,21.3708226936792,-2.03899763425965));
#51460=CARTESIAN_POINT('Ctrl Pts',(20.1808452608424,21.3245934161189,-2.04318236161637));
#51461=CARTESIAN_POINT('Ctrl Pts',(20.2484841862935,21.2749616395337,-2.04736708897308));
#51462=CARTESIAN_POINT('Ctrl Pts',(20.2636199524707,21.2638553873226,-2.04830351802431));
#51463=CARTESIAN_POINT('Ctrl Pts',(20.2786385693017,21.2525789442955,-2.04923994707554));
#51464=CARTESIAN_POINT('Ctrl Pts',(20.2935358855687,21.2411349269503,-2.05017637612677));
#51465=CARTESIAN_POINT('Ctrl Pts',(20.2935358855687,21.2411349269503,-1.25003886315632));
#51466=CARTESIAN_POINT('Ctrl Pts',(20.3601834809874,21.1899366960531,-1.25422273027566));
#51467=CARTESIAN_POINT('Ctrl Pts',(20.4242257520562,21.1355156975242,-1.258406597395));
#51468=CARTESIAN_POINT('Ctrl Pts',(20.4853525076874,21.0781808679978,-1.26259046451434));
#51469=CARTESIAN_POINT('Ctrl Pts',(20.5299990646909,21.0363039074377,-1.26564633194767));
#51470=CARTESIAN_POINT('Ctrl Pts',(20.5730910160661,20.9928733025549,-1.26870219938101));
#51471=CARTESIAN_POINT('Ctrl Pts',(20.6145211583455,20.948020487218,-1.27175806681434));
#51472=CARTESIAN_POINT('Ctrl Pts',(20.6712532036771,20.8866016309711,-1.27594259528124));
#51473=CARTESIAN_POINT('Ctrl Pts',(20.7250787538107,20.8222861461377,-1.28012712374813));
#51474=CARTESIAN_POINT('Ctrl Pts',(20.7756877958407,20.7553804402786,-1.28431165221502));
#51475=CARTESIAN_POINT('Ctrl Pts',(20.8262247807555,20.6885699947122,-1.2884902227535));
#51476=CARTESIAN_POINT('Ctrl Pts',(20.8735540790342,20.6191770173187,-1.29266879329197));
#51477=CARTESIAN_POINT('Ctrl Pts',(20.9174037187929,20.5475433778076,-1.29684736383044));
#51478=CARTESIAN_POINT('Ctrl Pts',(20.9620407606536,20.4746234226361,-1.30110096839983));
#51479=CARTESIAN_POINT('Ctrl Pts',(21.0030716129383,20.399381892885,-1.30535457296922));
#51480=CARTESIAN_POINT('Ctrl Pts',(21.0402535236503,20.3222131589622,-1.30960817753861));
#51481=CARTESIAN_POINT('Ctrl Pts',(21.0767133936984,20.2465429753506,-1.31377918077288));
#51482=CARTESIAN_POINT('Ctrl Pts',(21.1094722631679,20.1690202013163,-1.31795018400715));
#51483=CARTESIAN_POINT('Ctrl Pts',(21.1383468618206,20.0900427566697,-1.32212118724142));
#51484=CARTESIAN_POINT('Ctrl Pts',(21.1672117644678,20.0110918324171,-1.32629078986506));
#51485=CARTESIAN_POINT('Ctrl Pts',(21.1921948288651,19.9306876393951,-1.3304603924887));
#51486=CARTESIAN_POINT('Ctrl Pts',(21.2131612203808,19.8492473214673,-1.33462999511234));
#51487=CARTESIAN_POINT('Ctrl Pts',(21.2341268617413,19.7678099173871,-1.33879944855205));
#51488=CARTESIAN_POINT('Ctrl Pts',(21.2510760020805,19.6853369078528,-1.34296890199176));
#51489=CARTESIAN_POINT('Ctrl Pts',(21.2639242673564,19.6022584841778,-1.34713835543148));
#51490=CARTESIAN_POINT('Ctrl Pts',(21.2772250225956,19.5162542061506,-1.3514546486035));
#51491=CARTESIAN_POINT('Ctrl Pts',(21.2861305797708,19.4296015962165,-1.35577094177553));
#51492=CARTESIAN_POINT('Ctrl Pts',(21.290605703432,19.342784965678,-1.36008723494755));
#51493=CARTESIAN_POINT('Ctrl Pts',(21.2949348020335,19.2588011962232,-1.36426268576165));
#51494=CARTESIAN_POINT('Ctrl Pts',(21.2951181996998,19.1746644168246,-1.36843813657575));
#51495=CARTESIAN_POINT('Ctrl Pts',(21.2911771388899,19.0908123120325,-1.37261358738984));
#51496=CARTESIAN_POINT('Ctrl Pts',(21.287036673876,19.0027175773967,-1.37700030174083));
#51497=CARTESIAN_POINT('Ctrl Pts',(21.2783434334409,18.9149376655593,-1.38138701609182));
#51498=CARTESIAN_POINT('Ctrl Pts',(21.2651832584911,18.8279708732557,-1.38577373044281));
#51499=CARTESIAN_POINT('Ctrl Pts',(21.2520230835413,18.7410040809521,-1.3901604447938));
#51500=CARTESIAN_POINT('Ctrl Pts',(21.2343961650043,18.6548509616386,-1.39454715914479));
#51501=CARTESIAN_POINT('Ctrl Pts',(21.2124488481584,18.5699919602204,-1.39893387349578));
#51502=CARTESIAN_POINT('Ctrl Pts',(21.1915123905031,18.489041432083,-1.40311854262417));
#51503=CARTESIAN_POINT('Ctrl Pts',(21.1665668243994,18.4089670901725,-1.40730321175256));
#51504=CARTESIAN_POINT('Ctrl Pts',(21.1377020191448,18.3301954795987,-1.41148788088095));
#51505=CARTESIAN_POINT('Ctrl Pts',(21.1088782968446,18.251535983777,-1.41566659401657));
#51506=CARTESIAN_POINT('Ctrl Pts',(21.0761465724026,18.1741759645832,-1.4198453071522));
#51507=CARTESIAN_POINT('Ctrl Pts',(21.0396471231834,18.0985291719078,-1.42402402028782));
#51508=CARTESIAN_POINT('Ctrl Pts',(21.0024938354146,18.0215272686688,-1.42827758944988));
#51509=CARTESIAN_POINT('Ctrl Pts',(20.9614366236921,17.9463010448911,-1.43253115861194));
#51510=CARTESIAN_POINT('Ctrl Pts',(20.9166757000861,17.8732680431963,-1.436784727774));
#51511=CARTESIAN_POINT('Ctrl Pts',(20.8727820900014,17.8016501711454,-1.44095587732199));
#51512=CARTESIAN_POINT('Ctrl Pts',(20.825327269893,17.7321416952153,-1.44512702686999));
#51513=CARTESIAN_POINT('Ctrl Pts',(20.7745466544998,17.6651121157052,-1.44929817641799));
#51514=CARTESIAN_POINT('Ctrl Pts',(20.7237830774839,17.5981050265737,-1.45346792642368));
#51515=CARTESIAN_POINT('Ctrl Pts',(20.6696961989423,17.5335755483831,-1.45763767642937));
#51516=CARTESIAN_POINT('Ctrl Pts',(20.6125638140492,17.4718628586149,-1.46180742643506));
#51517=CARTESIAN_POINT('Ctrl Pts',(20.5554334612232,17.4101523638248,-1.46597702813235));
#51518=CARTESIAN_POINT('Ctrl Pts',(20.4952581305601,17.3512587952533,-1.47014662982965));
#51519=CARTESIAN_POINT('Ctrl Pts',(20.4323539003177,17.2954859621303,-1.47431623152694));
#51520=CARTESIAN_POINT('Ctrl Pts',(20.3672392271932,17.2377532820859,-1.47863235224779));
#51521=CARTESIAN_POINT('Ctrl Pts',(20.2992006896764,17.1833650979518,-1.48294847296865));
#51522=CARTESIAN_POINT('Ctrl Pts',(20.2286263825151,17.1326131311303,-1.48726459368951));
#51523=CARTESIAN_POINT('Ctrl Pts',(20.1603497799314,17.0835135082167,-1.49144019343698));
#51524=CARTESIAN_POINT('Ctrl Pts',(20.0897004104967,17.0378171816056,-1.49561579318445));
#51525=CARTESIAN_POINT('Ctrl Pts',(20.0170578177754,16.9957432121207,-1.49979139293192));
#51526=CARTESIAN_POINT('Ctrl Pts',(19.9407482759489,16.9515453770223,-1.50417777413947));
#51527=CARTESIAN_POINT('Ctrl Pts',(19.8622395019827,16.9113454968475,-1.50856415534702));
#51528=CARTESIAN_POINT('Ctrl Pts',(19.7819968173662,16.8753410628282,-1.51295053655457));
#51529=CARTESIAN_POINT('Ctrl Pts',(19.7017541327497,16.8393366288089,-1.51733691776211));
#51530=CARTESIAN_POINT('Ctrl Pts',(19.6197781058327,16.8075277799099,-1.52172329896966));
#51531=CARTESIAN_POINT('Ctrl Pts',(19.5365517913736,16.7800514974268,-1.52610968017721));
#51532=CARTESIAN_POINT('Ctrl Pts',(19.4571532093841,16.7538389001049,-1.53029432358246));
#51533=CARTESIAN_POINT('Ctrl Pts',(19.3763213117682,16.7314715386277,-1.53447896698771));
#51534=CARTESIAN_POINT('Ctrl Pts',(19.2944633944869,16.713104729289,-1.53866361039296));
#51535=CARTESIAN_POINT('Ctrl Pts',(19.2127219865111,16.6947640616392,-1.54284229774762));
#51536=CARTESIAN_POINT('Ctrl Pts',(19.1299579046074,16.6804127358414,-1.54702098510227));
#51537=CARTESIAN_POINT('Ctrl Pts',(19.0465949713152,16.6701567573129,-1.55119967245693));
#51538=CARTESIAN_POINT('Ctrl Pts',(18.9617380512092,16.6597169765107,-1.555453248057));
#51539=CARTESIAN_POINT('Ctrl Pts',(18.8762610609814,16.6535209330019,-1.55970682365707));
#51540=CARTESIAN_POINT('Ctrl Pts',(18.7906234644726,16.6516262908143,-1.56396039925714));
#51541=CARTESIAN_POINT('Ctrl Pts',(18.7066458766308,16.6497683745809,-1.5681315230761));
#51542=CARTESIAN_POINT('Ctrl Pts',(18.622514334468,16.6520466005142,-1.57230264689506));
#51543=CARTESIAN_POINT('Ctrl Pts',(18.5386669502935,16.6584630267727,-1.57647377071402));
#51544=CARTESIAN_POINT('Ctrl Pts',(18.4548476979935,16.6648773002377,-1.58064349506736));
#51545=CARTESIAN_POINT('Ctrl Pts',(18.3713128726456,16.6754269815325,-1.5848132194207));
#51546=CARTESIAN_POINT('Ctrl Pts',(18.2884980297119,16.6900620804015,-1.58898294377403));
#51547=CARTESIAN_POINT('Ctrl Pts',(18.2056861301165,16.7046966591217,-1.5931525199304));
#51548=CARTESIAN_POINT('Ctrl Pts',(18.1235946149204,16.7234162858241,-1.59732209608677));
#51549=CARTESIAN_POINT('Ctrl Pts',(18.0426500224206,16.7461196360673,-1.60149167224313));
#51550=CARTESIAN_POINT('Ctrl Pts',(17.9588599467863,16.7696210878046,-1.60580782346109));
#51551=CARTESIAN_POINT('Ctrl Pts',(17.8762994412694,16.7973914245208,-1.61012397467905));
#51552=CARTESIAN_POINT('Ctrl Pts',(17.7954238786636,16.8292622175275,-1.61444012589701));
#51553=CARTESIAN_POINT('Ctrl Pts',(17.7171824223145,16.8600949830688,-1.6186157006471));
#51554=CARTESIAN_POINT('Ctrl Pts',(17.6405182467689,16.8947649654851,-1.62279127539719));
#51555=CARTESIAN_POINT('Ctrl Pts',(17.5658209824087,16.9330716027804,-1.62696685014728));
#51556=CARTESIAN_POINT('Ctrl Pts',(17.4873515388115,16.9733127085343,-1.63135328959917));
#51557=CARTESIAN_POINT('Ctrl Pts',(17.4110533973333,17.0175671442341,-1.63573972905107));
#51558=CARTESIAN_POINT('Ctrl Pts',(17.3373445043261,17.0655505304473,-1.64012616850296));
#51559=CARTESIAN_POINT('Ctrl Pts',(17.2636356113189,17.1135339166605,-1.64451260795486));
#51560=CARTESIAN_POINT('Ctrl Pts',(17.1925163913081,17.1652458506637,-1.64889904740675));
#51561=CARTESIAN_POINT('Ctrl Pts',(17.1243635063082,17.2203542861233,-1.65328548685865));
#51562=CARTESIAN_POINT('Ctrl Pts',(17.0601943716838,17.27224146029,-1.65741552513525));
#51563=CARTESIAN_POINT('Ctrl Pts',(16.9984022161797,17.3273436089106,-1.66154556341186));
#51564=CARTESIAN_POINT('Ctrl Pts',(16.9393333495131,17.3854119814071,-1.66567560168847));
#51565=CARTESIAN_POINT('Ctrl Pts',(16.8791242534032,17.4446012704164,-1.66988536370976));
#51566=CARTESIAN_POINT('Ctrl Pts',(16.8217451257373,17.5068722664466,-1.67409512573104));
#51567=CARTESIAN_POINT('Ctrl Pts',(16.7675298311078,17.5719163917429,-1.67830488775233));
#51568=CARTESIAN_POINT('Ctrl Pts',(16.7144792339723,17.6355631857096,-1.6824242122078));
#51569=CARTESIAN_POINT('Ctrl Pts',(16.6644582224381,17.701864774228,-1.68654353666328));
#51570=CARTESIAN_POINT('Ctrl Pts',(16.6177431433907,17.7704942149182,-1.69066286111875));
#51571=CARTESIAN_POINT('Ctrl Pts',(16.5710563616802,17.8390820837981,-1.69477969032184));
#51572=CARTESIAN_POINT('Ctrl Pts',(16.5276718045391,17.9099946168291,-1.69889651952493));
#51573=CARTESIAN_POINT('Ctrl Pts',(16.4878244173549,17.9828732752973,-1.70301334872802));
#51574=CARTESIAN_POINT('Ctrl Pts',(16.4479884744815,18.0557310027567,-1.70712899556318));
#51575=CARTESIAN_POINT('Ctrl Pts',(16.4116879110196,18.1305533194009,-1.71124464239834));
#51576=CARTESIAN_POINT('Ctrl Pts',(16.3791125474012,18.206955635645,-1.7153602892335));
#51577=CARTESIAN_POINT('Ctrl Pts',(16.3452431867613,18.2863928948241,-1.71963942264732));
#51578=CARTESIAN_POINT('Ctrl Pts',(16.3154014151592,18.367537815818,-1.72391855606114));
#51579=CARTESIAN_POINT('Ctrl Pts',(16.2897454150196,18.4499352696373,-1.72819768947497));
#51580=CARTESIAN_POINT('Ctrl Pts',(16.265047031356,18.529257218353,-1.73231710318821));
#51581=CARTESIAN_POINT('Ctrl Pts',(16.2442275674438,18.6097393677812,-1.73643651690145));
#51582=CARTESIAN_POINT('Ctrl Pts',(16.2273766224859,18.690962267427,-1.74055593061469));
#51583=CARTESIAN_POINT('Ctrl Pts',(16.2105163819041,18.7722299727216,-1.74467761675363));
#51584=CARTESIAN_POINT('Ctrl Pts',(16.1976290874525,18.8542387741595,-1.74879930289257));
#51585=CARTESIAN_POINT('Ctrl Pts',(16.1887526583662,18.9365624480759,-1.75292098903151));
#51586=CARTESIAN_POINT('Ctrl Pts',(16.1798641545679,19.018998107865,-1.75704828194913));
#51587=CARTESIAN_POINT('Ctrl Pts',(16.1749974202386,19.1017490235124,-1.76117557486675));
#51588=CARTESIAN_POINT('Ctrl Pts',(16.1741383212113,19.1843882456639,-1.76530286778437));
#51589=CARTESIAN_POINT('Ctrl Pts',(16.1740406969644,19.1937790045501,-1.76577187525603));
#51590=CARTESIAN_POINT('Ctrl Pts',(16.173994768433,19.2031683266851,-1.7662408827277));
#51591=CARTESIAN_POINT('Ctrl Pts',(16.1740004726294,19.2125555906437,-1.76670989019937));
#51592=CARTESIAN_POINT('Origin',(18.734,19.211,1.76670989022852));
#51593=CARTESIAN_POINT('',(20.2910039445873,21.2378222631174,-0.450077510930245));
#51594=CARTESIAN_POINT('',(20.2957383200499,21.2439676837843,-0.516748669299169));
#51595=CARTESIAN_POINT('',(20.2935358855687,21.2411349269503,1.76670989022852));
#51596=CARTESIAN_POINT('',(16.1765334933267,19.2078568329122,-0.166709890228504));
#51597=CARTESIAN_POINT('Ctrl Pts',(16.1765334933267,19.2078568329122,-0.166709890228504));
#51598=CARTESIAN_POINT('Ctrl Pts',(16.1810511662408,19.7963216342631,-0.195923797939959));
#51599=CARTESIAN_POINT('Ctrl Pts',(16.6739009423912,21.2477390833877,-0.267529641211891));
#51600=CARTESIAN_POINT('Ctrl Pts',(18.6725570476074,22.0506151623629,-0.361985514779138));
#51601=CARTESIAN_POINT('Ctrl Pts',(19.9247548523317,21.5178475229395,-0.427227480634931));
#51602=CARTESIAN_POINT('Ctrl Pts',(20.2910039445873,21.2378222631174,-0.450077510930245));
#51603=CARTESIAN_POINT('',(18.0722627314315,16.7380050975816,0.));
#51604=CARTESIAN_POINT('Ctrl Pts',(18.0722627314315,16.7380050975816,1.38777878078145E-15));
#51605=CARTESIAN_POINT('Ctrl Pts',(17.2488902483963,16.9583275322964,-0.0423919355604767));
#51606=CARTESIAN_POINT('Ctrl Pts',(16.3345567825823,17.8262089039162,-0.0979618989699788));
#51607=CARTESIAN_POINT('Ctrl Pts',(16.1744956276614,18.942407731855,-0.153531862379481));
#51608=CARTESIAN_POINT('Ctrl Pts',(16.1765334933267,19.2078568329122,-0.166709890228504));
#51609=CARTESIAN_POINT('',(19.395767528315,16.7380131948456,-1.73172587381032E-11));
#51610=CARTESIAN_POINT('Origin',(18.734,19.211,0.));
#51611=CARTESIAN_POINT('',(16.1740007446525,19.2129525932361,-0.233290109771496));
#51612=CARTESIAN_POINT('Ctrl Pts',(19.395767528315,16.7380131948456,-1.73172587381032E-11));
#51613=CARTESIAN_POINT('Ctrl Pts',(19.3150528289901,16.7164140633987,-0.0041815967549353));
#51614=CARTESIAN_POINT('Ctrl Pts',(19.2331283959629,16.6987302550736,-0.00836319349255328));
#51615=CARTESIAN_POINT('Ctrl Pts',(19.1504091887632,16.685093551314,-0.0125447902301714));
#51616=CARTESIAN_POINT('Ctrl Pts',(19.0678077744006,16.6714762663337,-0.0167204323393492));
#51617=CARTESIAN_POINT('Ctrl Pts',(18.9844142845817,16.6618947132319,-0.0208960744485263));
#51618=CARTESIAN_POINT('Ctrl Pts',(18.9006573782918,16.6564305023623,-0.0250717165577041));
#51619=CARTESIAN_POINT('Ctrl Pts',(18.8165042143108,16.6509404400653,-0.0292671138175207));
#51620=CARTESIAN_POINT('Ctrl Pts',(18.7319846403618,16.6496069070114,-0.0334625110773381));
#51621=CARTESIAN_POINT('Ctrl Pts',(18.6475423744123,16.6524603620468,-0.0376579083371547));
#51622=CARTESIAN_POINT('Ctrl Pts',(18.5636493738553,16.6552952564233,-0.0418260161051873));
#51623=CARTESIAN_POINT('Ctrl Pts',(18.4798331446954,16.6622628172183,-0.0459941238732202));
#51624=CARTESIAN_POINT('Ctrl Pts',(18.3965307038144,16.6733407490106,-0.0501622316412529));
#51625=CARTESIAN_POINT('Ctrl Pts',(18.3132563453466,16.6844149462778,-0.0543289342820943));
#51626=CARTESIAN_POINT('Ctrl Pts',(18.2304958875343,16.6995967018794,-0.0584956369229356));
#51627=CARTESIAN_POINT('Ctrl Pts',(18.1486808927462,16.718811896609,-0.0626623395637771));
#51628=CARTESIAN_POINT('Ctrl Pts',(18.0668688404716,16.7380264002553,-0.0668288923472635));
#51629=CARTESIAN_POINT('Ctrl Pts',(17.9860026319441,16.7612739482847,-0.0709954451307501));
#51630=CARTESIAN_POINT('Ctrl Pts',(17.9065019549449,16.7884296737907,-0.0751619979142366));
#51631=CARTESIAN_POINT('Ctrl Pts',(17.8260462587421,16.8159116133658,-0.0793786023208257));
#51632=CARTESIAN_POINT('Ctrl Pts',(17.7469895837595,16.8473961156675,-0.0835952067274143));
#51633=CARTESIAN_POINT('Ctrl Pts',(17.6697476948766,16.8827029761992,-0.0878118111340034));
#51634=CARTESIAN_POINT('Ctrl Pts',(17.5933154552392,16.9176397503257,-0.0919842171059645));
#51635=CARTESIAN_POINT('Ctrl Pts',(17.5186605203447,16.9563188567597,-0.0961566230779257));
#51636=CARTESIAN_POINT('Ctrl Pts',(17.4461607527195,16.9985194750769,-0.100329029049887));
#51637=CARTESIAN_POINT('Ctrl Pts',(17.3725089964354,17.041390642215,-0.10456773267379));
#51638=CARTESIAN_POINT('Ctrl Pts',(17.3010819091514,17.0878959373098,-0.108806436297694));
#51639=CARTESIAN_POINT('Ctrl Pts',(17.2322432877688,17.1377593537487,-0.113045139921597));
#51640=CARTESIAN_POINT('Ctrl Pts',(17.1634046663863,17.1876227701875,-0.1172838435455));
#51641=CARTESIAN_POINT('Ctrl Pts',(17.0971548535428,17.2408439496524,-0.121522547169403));
#51642=CARTESIAN_POINT('Ctrl Pts',(17.0338195264424,17.2971070151826,-0.125761250793306));
#51643=CARTESIAN_POINT('Ctrl Pts',(16.9721381147478,17.3519008477408,-0.129889266471862));
#51644=CARTESIAN_POINT('Ctrl Pts',(16.9129812130569,17.4097927309776,-0.134017282150418));
#51645=CARTESIAN_POINT('Ctrl Pts',(16.8566825236081,17.4705175689386,-0.138145297828974));
#51646=CARTESIAN_POINT('Ctrl Pts',(16.8004749046566,17.5311441765279,-0.142266635901988));
#51647=CARTESIAN_POINT('Ctrl Pts',(16.7471166302611,17.5945942890769,-0.146387973975001));
#51648=CARTESIAN_POINT('Ctrl Pts',(16.6969071786038,17.6605636623788,-0.150509312048014));
#51649=CARTESIAN_POINT('Ctrl Pts',(16.6467433533799,17.7264730878598,-0.154626904970446));
#51650=CARTESIAN_POINT('Ctrl Pts',(16.5997229600923,17.7948968581842,-0.158744497892878));
#51651=CARTESIAN_POINT('Ctrl Pts',(16.5561068210809,17.8654958932736,-0.16286209081531));
#51652=CARTESIAN_POINT('Ctrl Pts',(16.5125163943093,17.9360533093806,-0.16697725636706));
#51653=CARTESIAN_POINT('Ctrl Pts',(16.4723264875143,18.0087830434683,-0.171092421918811));
#51654=CARTESIAN_POINT('Ctrl Pts',(16.4357550862559,18.0833163934643,-0.175207587470561));
#51655=CARTESIAN_POINT('Ctrl Pts',(16.3991935732988,18.1578295908767,-0.179321640349689));
#51656=CARTESIAN_POINT('Ctrl Pts',(16.3662488306646,18.2341450104433,-0.183435693228817));
#51657=CARTESIAN_POINT('Ctrl Pts',(16.3370925482536,18.3118700495687,-0.187549746107944));
#51658=CARTESIAN_POINT('Ctrl Pts',(16.3079200305285,18.3896383689178,-0.191666089846375));
#51659=CARTESIAN_POINT('Ctrl Pts',(16.2825403575632,18.4688174331029,-0.195782433584806));
#51660=CARTESIAN_POINT('Ctrl Pts',(16.2610764229501,18.5489962371172,-0.199898777323237));
#51661=CARTESIAN_POINT('Ctrl Pts',(16.239606571517,18.6291971434892,-0.204016255786767));
#51662=CARTESIAN_POINT('Ctrl Pts',(16.2220547120702,18.7103978759457,-0.208133734250297));
#51663=CARTESIAN_POINT('Ctrl Pts',(16.2084928021298,18.7921761784404,-0.212251212713827));
#51664=CARTESIAN_POINT('Ctrl Pts',(16.1949128183452,18.874063466196,-0.21637417850653));
#51665=CARTESIAN_POINT('Ctrl Pts',(16.1853334600005,18.9565293904166,-0.220497144299234));
#51666=CARTESIAN_POINT('Ctrl Pts',(16.1797748247972,19.0391461249782,-0.224620110091938));
#51667=CARTESIAN_POINT('Ctrl Pts',(16.1758784899859,19.0970564657531,-0.227510109985124));
#51668=CARTESIAN_POINT('Ctrl Pts',(16.1739565734894,19.1550408159346,-0.230400109878309));
#51669=CARTESIAN_POINT('Ctrl Pts',(16.1740007446525,19.2129525932361,-0.233290109771496));
#51670=CARTESIAN_POINT('Ctrl Pts',(16.1719919784605,19.2129541253863,-0.233290109771496));
#51671=CARTESIAN_POINT('Ctrl Pts',(16.1708576353774,19.3442909950989,-0.239839092339242));
#51672=CARTESIAN_POINT('Ctrl Pts',(16.2398215309513,20.3246257991586,-0.288780010467465));
#51673=CARTESIAN_POINT('Ctrl Pts',(17.5061738855977,21.978179087,-0.380112864156167));
#51674=CARTESIAN_POINT('Ctrl Pts',(19.5043144350046,21.8141354816799,-0.468050068097647));
#51675=CARTESIAN_POINT('Ctrl Pts',(20.2458873728542,21.2827381199421,-0.513595336478648));
#51676=CARTESIAN_POINT('Ctrl Pts',(20.2957383200499,21.2439676837843,-0.516748669299169));
#51677=CARTESIAN_POINT('Origin',(18.734,-18.952,1.76670989022851));
#51678=CARTESIAN_POINT('',(20.2955778924961,-16.9192440454753,-21.2501821980133));
#51679=CARTESIAN_POINT('',(20.2916907304467,-16.9243022127158,-21.3166133950378));
#51680=CARTESIAN_POINT('',(20.293535888361,-16.9218650751948,1.76670989022851));
#51681=CARTESIAN_POINT('',(16.1765333501007,-18.9488555363839,-21.8332901097715));
#51682=CARTESIAN_POINT('Ctrl Pts',(20.2916907304466,-16.9243022127157,-21.3166133950378));
#51683=CARTESIAN_POINT('Ctrl Pts',(20.5461545344098,-17.1171758877203,-21.3324492522228));
#51684=CARTESIAN_POINT('Ctrl Pts',(21.3518775433702,-17.9919927123694,-21.3906770449683));
#51685=CARTESIAN_POINT('Ctrl Pts',(21.4520480948179,-20.2843429650063,-21.4912967732743));
#51686=CARTESIAN_POINT('Ctrl Pts',(19.0860574215255,-21.9577201113934,-21.6184725799557));
#51687=CARTESIAN_POINT('Ctrl Pts',(16.6739013977444,-20.9887406839414,-21.7324703587881));
#51688=CARTESIAN_POINT('Ctrl Pts',(16.1810511496244,-19.5373209132916,-21.80407620206));
#51689=CARTESIAN_POINT('Ctrl Pts',(16.1765333501007,-18.9488555363839,-21.8332901097715));
#51690=CARTESIAN_POINT('',(18.0722627314314,-16.4790050975816,-22.));
#51691=CARTESIAN_POINT('Ctrl Pts',(16.1765333501007,-18.9488555363839,-21.8332901097715));
#51692=CARTESIAN_POINT('Ctrl Pts',(16.1744954273233,-18.6834061757001,-21.8464681376205));
#51693=CARTESIAN_POINT('Ctrl Pts',(16.3345563979949,-17.5672065717878,-21.90203810103));
#51694=CARTESIAN_POINT('Ctrl Pts',(17.2488902483963,-16.6993275322964,-21.9576080644395));
#51695=CARTESIAN_POINT('Ctrl Pts',(18.0722627314314,-16.4790050975816,-22.));
#51696=CARTESIAN_POINT('',(19.3957679668415,-16.4790133121946,-21.9999999999819));
#51697=CARTESIAN_POINT('Origin',(18.734,-18.952,-22.));
#51698=CARTESIAN_POINT('',(16.1740007447319,-18.9539526972956,-21.7667098902285));
#51699=CARTESIAN_POINT('Ctrl Pts',(16.1740007447319,-18.9539526972956,-21.7667098902285));
#51700=CARTESIAN_POINT('Ctrl Pts',(16.1739377135638,-18.8713184130896,-21.770833628584));
#51701=CARTESIAN_POINT('Ctrl Pts',(16.1778799218946,-18.788536175973,-21.7749573669396));
#51702=CARTESIAN_POINT('Ctrl Pts',(16.1858438033836,-18.7060325272615,-21.7790811052951));
#51703=CARTESIAN_POINT('Ctrl Pts',(16.1937978807278,-18.6236304468261,-21.7831997670146));
#51704=CARTESIAN_POINT('Ctrl Pts',(16.2057637513171,-18.5415067419993,-21.787318428734));
#51705=CARTESIAN_POINT('Ctrl Pts',(16.2217058130157,-18.4600874894405,-21.7914370904535));
#51706=CARTESIAN_POINT('Ctrl Pts',(16.2376371830466,-18.3787228413373,-21.7955529899605));
#51707=CARTESIAN_POINT('Ctrl Pts',(16.2575393635618,-18.2980621716067,-21.7996688894674));
#51708=CARTESIAN_POINT('Ctrl Pts',(16.2813251279379,-18.2185247298273,-21.8037847889744));
#51709=CARTESIAN_POINT('Ctrl Pts',(16.3051025309066,-18.1390152478366,-21.8078992416196));
#51710=CARTESIAN_POINT('Ctrl Pts',(16.3327606725193,-18.060628663487,-21.8120136942648));
#51711=CARTESIAN_POINT('Ctrl Pts',(16.3641619710533,-17.9837708346893,-21.81612814691));
#51712=CARTESIAN_POINT('Ctrl Pts',(16.3955622513427,-17.9069154981478,-21.8202424661365));
#51713=CARTESIAN_POINT('Ctrl Pts',(16.4307052665747,-17.8315892564416,-21.824356785363));
#51714=CARTESIAN_POINT('Ctrl Pts',(16.4694052036476,-17.7581782342687,-21.8284711045895));
#51715=CARTESIAN_POINT('Ctrl Pts',(16.5081407912399,-17.6846995856017,-21.8325892139415));
#51716=CARTESIAN_POINT('Ctrl Pts',(16.5504396217143,-17.6131400990191,-21.8367073232935));
#51717=CARTESIAN_POINT('Ctrl Pts',(16.5960701372503,-17.543860837146,-21.8408254326455));
#51718=CARTESIAN_POINT('Ctrl Pts',(16.6417225438979,-17.4745483387418,-21.8449455176489));
#51719=CARTESIAN_POINT('Ctrl Pts',(16.6907095365088,-17.407518624288,-21.8490656026523));
#51720=CARTESIAN_POINT('Ctrl Pts',(16.7427579736743,-17.343101248495,-21.8531856876557));
#51721=CARTESIAN_POINT('Ctrl Pts',(16.794892440757,-17.2785773983907,-21.8573125826728));
#51722=CARTESIAN_POINT('Ctrl Pts',(16.8500981395581,-17.2166748608617,-21.8614394776899));
#51723=CARTESIAN_POINT('Ctrl Pts',(16.9080639839603,-17.1576874114779,-21.865566372707));
#51724=CARTESIAN_POINT('Ctrl Pts',(16.9486676843771,-17.1163681009799,-21.8684571648736));
#51725=CARTESIAN_POINT('Ctrl Pts',(16.9906249225133,-17.0764783454379,-21.8713479570401));
#51726=CARTESIAN_POINT('Ctrl Pts',(17.0338195571032,-17.0381069879455,-21.8742387492067));
#51727=CARTESIAN_POINT('Ctrl Pts',(17.0962945700832,-16.9826081724059,-21.8784198767899));
#51728=CARTESIAN_POINT('Ctrl Pts',(17.1616053466634,-16.9300690778322,-21.8826010043731));
#51729=CARTESIAN_POINT('Ctrl Pts',(17.2294395634032,-16.8807931313779,-21.8867821319562));
#51730=CARTESIAN_POINT('Ctrl Pts',(17.2971787572344,-16.8315862112052,-21.8909574025704));
#51731=CARTESIAN_POINT('Ctrl Pts',(17.3674340003121,-16.7856336283223,-21.8951326731846));
#51732=CARTESIAN_POINT('Ctrl Pts',(17.4398582963668,-16.7432000428021,-21.8993079437988));
#51733=CARTESIAN_POINT('Ctrl Pts',(17.5126335322061,-16.7005608407393,-21.9035034461398));
#51734=CARTESIAN_POINT('Ctrl Pts',(17.5875985480893,-16.6614751468356,-21.9076989484807));
#51735=CARTESIAN_POINT('Ctrl Pts',(17.6643699161775,-16.6261686467455,-21.9118944508217));
#51736=CARTESIAN_POINT('Ctrl Pts',(17.7406375998075,-16.5910937868593,-21.9160624271542));
#51737=CARTESIAN_POINT('Ctrl Pts',(17.8186875806148,-16.5597488751243,-21.9202304034868));
#51738=CARTESIAN_POINT('Ctrl Pts',(17.8981189457525,-16.5323093455671,-21.9243983798194));
#51739=CARTESIAN_POINT('Ctrl Pts',(17.9775252548951,-16.5048784715922,-21.9285650413968));
#51740=CARTESIAN_POINT('Ctrl Pts',(18.0583116477557,-16.4813506834989,-21.9327317029742));
#51741=CARTESIAN_POINT('Ctrl Pts',(18.140058939298,-16.4618526115083,-21.9368983645517));
#51742=CARTESIAN_POINT('Ctrl Pts',(18.221805062827,-16.442354818108,-21.9410649665954));
#51743=CARTESIAN_POINT('Ctrl Pts',(18.3045116092593,-16.4268867321271,-21.9452315686392));
#51744=CARTESIAN_POINT('Ctrl Pts',(18.3877473464946,-16.4155242757045,-21.949398170683));
#51745=CARTESIAN_POINT('Ctrl Pts',(18.4719862643407,-16.4040248757484,-21.9536149897912));
#51746=CARTESIAN_POINT('Ctrl Pts',(18.5567667383604,-16.3967308160666,-21.9578318088995));
#51747=CARTESIAN_POINT('Ctrl Pts',(18.6416363028402,-16.3936667637997,-21.9620486280077));
#51748=CARTESIAN_POINT('Ctrl Pts',(18.7256174343068,-16.3906347866968,-21.9662213045387));
#51749=CARTESIAN_POINT('Ctrl Pts',(18.8096853344826,-16.3917446006535,-21.9703939810697));
#51750=CARTESIAN_POINT('Ctrl Pts',(18.8934033137616,-16.3969675963773,-21.9745666576007));
#51751=CARTESIAN_POINT('Ctrl Pts',(18.9784497667458,-16.4022734728939,-21.9788055479976));
#51752=CARTESIAN_POINT('Ctrl Pts',(19.0631346044502,-16.4118241506696,-21.9830444383944));
#51753=CARTESIAN_POINT('Ctrl Pts',(19.1470091266727,-16.4255353829343,-21.9872833287913));
#51754=CARTESIAN_POINT('Ctrl Pts',(19.2308836488952,-16.439246615199,-21.9915222191882));
#51755=CARTESIAN_POINT('Ctrl Pts',(19.3139473893182,-16.4571182338667,-21.9957611095851));
#51756=CARTESIAN_POINT('Ctrl Pts',(19.3957679668415,-16.4790133121946,-21.9999999999819));
#51757=CARTESIAN_POINT('Ctrl Pts',(20.2955778924961,-16.9192440454753,-21.2501821980133));
#51758=CARTESIAN_POINT('Ctrl Pts',(20.9031379978352,-17.3928060279424,-21.2886333061692));
#51759=CARTESIAN_POINT('Ctrl Pts',(21.7186680704123,-19.0034153201252,-21.3694763498856));
#51760=CARTESIAN_POINT('Ctrl Pts',(20.3959081902549,-21.4819377002129,-21.4927113291624));
#51761=CARTESIAN_POINT('Ctrl Pts',(17.5061736134544,-21.7191789276414,-21.6198871358439));
#51762=CARTESIAN_POINT('Ctrl Pts',(16.2398215663958,-20.0656261776283,-21.7112199895325));
#51763=CARTESIAN_POINT('Ctrl Pts',(16.1708575232621,-19.0852911366623,-21.7601609076608));
#51764=CARTESIAN_POINT('Ctrl Pts',(16.1719918438157,-18.9539542296302,-21.7667098902285));
#51765=CARTESIAN_POINT('Origin',(18.734,-18.952,1.76670989022851));
#51766=CARTESIAN_POINT('',(20.2940725979672,-16.9211546778498,-20.4499991793503));
#51767=CARTESIAN_POINT('',(20.293535888361,-16.9218650751948,-20.5167505018104));
#51768=CARTESIAN_POINT('',(20.293535888361,-16.9218650751948,1.76670989022851));
#51769=CARTESIAN_POINT('',(16.1740711621187,-18.953341697584,-21.0332900817674));
#51770=CARTESIAN_POINT('Ctrl Pts',(20.293535888361,-16.9218650751948,-20.5167505018104));
#51771=CARTESIAN_POINT('Ctrl Pts',(20.3601729838807,-16.9730552402864,-20.5209209411032));
#51772=CARTESIAN_POINT('Ctrl Pts',(20.4243268584381,-17.0275603845044,-20.525091380396));
#51773=CARTESIAN_POINT('Ctrl Pts',(20.4856569049576,-17.0851046929958,-20.5292618196889));
#51774=CARTESIAN_POINT('Ctrl Pts',(20.5469737360019,-17.1426366017675,-20.5334313603302));
#51775=CARTESIAN_POINT('Ctrl Pts',(20.6054676124936,-17.2032060591384,-20.5376009009716));
#51776=CARTESIAN_POINT('Ctrl Pts',(20.660832945591,-17.2664986503164,-20.5417704416129));
#51777=CARTESIAN_POINT('Ctrl Pts',(20.7162029558448,-17.3297965883304,-20.545940334489));
#51778=CARTESIAN_POINT('Ctrl Pts',(20.7684435960241,-17.3958177698225,-20.5501102273651));
#51779=CARTESIAN_POINT('Ctrl Pts',(20.8172888275803,-17.4642138389946,-20.5542801202412));
#51780=CARTESIAN_POINT('Ctrl Pts',(20.8661854276987,-17.5326818375574,-20.5584543984257));
#51781=CARTESIAN_POINT('Ctrl Pts',(20.9116792213078,-17.6035293356889,-20.5626286766101));
#51782=CARTESIAN_POINT('Ctrl Pts',(20.9535471879616,-17.6763784728957,-20.5668029547945));
#51783=CARTESIAN_POINT('Ctrl Pts',(20.9954381188789,-17.7492675673043,-20.5709795225391));
#51784=CARTESIAN_POINT('Ctrl Pts',(21.0336990535097,-17.8241600770645,-20.5751560902836));
#51785=CARTESIAN_POINT('Ctrl Pts',(21.0681538146031,-17.9006551613416,-20.5793326580281));
#51786=CARTESIAN_POINT('Ctrl Pts',(21.102668197055,-17.9772826145772,-20.5835164530072));
#51787=CARTESIAN_POINT('Ctrl Pts',(21.1333630832728,-18.0555177524356,-20.5877002479864));
#51788=CARTESIAN_POINT('Ctrl Pts',(21.1601112339645,-18.1349416909233,-20.5918840429655));
#51789=CARTESIAN_POINT('Ctrl Pts',(21.1796790948325,-18.1930450191058,-20.5949447374784));
#51790=CARTESIAN_POINT('Ctrl Pts',(21.1971357843348,-18.251784208033,-20.5980054319913));
#51791=CARTESIAN_POINT('Ctrl Pts',(21.2124488472332,-18.310991956643,-20.6010661265042));
#51792=CARTESIAN_POINT('Ctrl Pts',(21.2333845648802,-18.3919396230659,-20.6052506476905));
#51793=CARTESIAN_POINT('Ctrl Pts',(21.2503893834069,-18.4740647142243,-20.6094351688768));
#51794=CARTESIAN_POINT('Ctrl Pts',(21.26333508953,-18.556950629829,-20.6136196900631));
#51795=CARTESIAN_POINT('Ctrl Pts',(21.2762623681317,-18.6397185617596,-20.617798254807));
#51796=CARTESIAN_POINT('Ctrl Pts',(21.2851419407115,-18.7232447163151,-20.6219768195509));
#51797=CARTESIAN_POINT('Ctrl Pts',(21.2898958840996,-18.8070992420912,-20.6261553842948));
#51798=CARTESIAN_POINT('Ctrl Pts',(21.2947352019821,-18.8924596835152,-20.6304089904986));
#51799=CARTESIAN_POINT('Ctrl Pts',(21.2952991221814,-18.9781599402378,-20.6346625967024));
#51800=CARTESIAN_POINT('Ctrl Pts',(21.291560298641,-19.0637377233315,-20.6389162029062));
#51801=CARTESIAN_POINT('Ctrl Pts',(21.2878940830978,-19.1476535848685,-20.6430872040273));
#51802=CARTESIAN_POINT('Ctrl Pts',(21.2800907694637,-19.2314512062992,-20.6472582051485));
#51803=CARTESIAN_POINT('Ctrl Pts',(21.2681770980697,-19.3146933079329,-20.6514292062697));
#51804=CARTESIAN_POINT('Ctrl Pts',(21.2562674233252,-19.3979074845465,-20.6555988081555));
#51805=CARTESIAN_POINT('Ctrl Pts',(21.2402501944417,-19.4805660564334,-20.6597684100413));
#51806=CARTESIAN_POINT('Ctrl Pts',(21.2202039195676,-19.5622377162439,-20.6639380119271));
#51807=CARTESIAN_POINT('Ctrl Pts',(21.2001583553192,-19.6439064808543,-20.6681074660036));
#51808=CARTESIAN_POINT('Ctrl Pts',(21.1760841395508,-19.7245879563529,-20.6722769200801));
#51809=CARTESIAN_POINT('Ctrl Pts',(21.1481104108274,-19.803863207525,-20.6764463741567));
#51810=CARTESIAN_POINT('Ctrl Pts',(21.1191514853748,-19.8859304253645,-20.6807626707424));
#51811=CARTESIAN_POINT('Ctrl Pts',(21.0860134227951,-19.9664900212761,-20.6850789673282));
#51812=CARTESIAN_POINT('Ctrl Pts',(21.0488942544675,-20.0450986188966,-20.6893952639139));
#51813=CARTESIAN_POINT('Ctrl Pts',(21.012986292885,-20.1211422004361,-20.6935707187789));
#51814=CARTESIAN_POINT('Ctrl Pts',(20.973353301723,-20.1953597550486,-20.697746173644));
#51815=CARTESIAN_POINT('Ctrl Pts',(20.9302210187628,-20.2673757017462,-20.701921628509));
#51816=CARTESIAN_POINT('Ctrl Pts',(20.8849064017287,-20.3430353891309,-20.7063083459551));
#51817=CARTESIAN_POINT('Ctrl Pts',(20.8357293771903,-20.416264321532,-20.7106950634012));
#51818=CARTESIAN_POINT('Ctrl Pts',(20.7830012667822,-20.486664070318,-20.7150817808473));
#51819=CARTESIAN_POINT('Ctrl Pts',(20.730273156374,-20.5570638191041,-20.7194684982935));
#51820=CARTESIAN_POINT('Ctrl Pts',(20.6739943901059,-20.6246339869631,-20.7238552157396));
#51821=CARTESIAN_POINT('Ctrl Pts',(20.6145211534102,-20.689020492561,-20.7282419331857));
#51822=CARTESIAN_POINT('Ctrl Pts',(20.5577862400574,-20.7504424534151,-20.7324266732139));
#51823=CARTESIAN_POINT('Ctrl Pts',(20.4979333332223,-20.809196146077,-20.7366114132421));
#51824=CARTESIAN_POINT('Ctrl Pts',(20.4352433664353,-20.8649482502566,-20.7407961532704));
#51825=CARTESIAN_POINT('Ctrl Pts',(20.3726426387416,-20.9206209913821,-20.7449749363261));
#51826=CARTESIAN_POINT('Ctrl Pts',(20.3072132137399,-20.9733003279932,-20.7491537193819));
#51827=CARTESIAN_POINT('Ctrl Pts',(20.2392743864999,-21.022688055055,-20.7533325024377));
#51828=CARTESIAN_POINT('Ctrl Pts',(20.1701199698419,-21.0729594476264,-20.7575860539972));
#51829=CARTESIAN_POINT('Ctrl Pts',(20.0983657941174,-21.1198199254428,-20.7618396055568));
#51830=CARTESIAN_POINT('Ctrl Pts',(20.0243857323821,-21.1629963052128,-20.7660931571163));
#51831=CARTESIAN_POINT('Ctrl Pts',(19.9518376847091,-21.2053369303006,-20.7702643737129));
#51832=CARTESIAN_POINT('Ctrl Pts',(19.8771495707328,-21.2441345685215,-20.7744355903094));
#51833=CARTESIAN_POINT('Ctrl Pts',(19.8007035796531,-21.2791749983951,-20.7786068069059));
#51834=CARTESIAN_POINT('Ctrl Pts',(19.7242832601421,-21.3142036612317,-20.7827766227531));
#51835=CARTESIAN_POINT('Ctrl Pts',(19.6461066537349,-21.3454774300037,-20.7869464386003));
#51836=CARTESIAN_POINT('Ctrl Pts',(19.5665789487914,-21.372828844431,-20.7911162544474));
#51837=CARTESIAN_POINT('Ctrl Pts',(19.4870540969431,-21.4001792776131,-20.7952859207004));
#51838=CARTESIAN_POINT('Ctrl Pts',(19.4061786782093,-21.4236074874285,-20.7994555869534));
#51839=CARTESIAN_POINT('Ctrl Pts',(19.3243748839096,-21.4429952823016,-20.8036252532064));
#51840=CARTESIAN_POINT('Ctrl Pts',(19.2396994033476,-21.4630636771966,-20.8079412937615));
#51841=CARTESIAN_POINT('Ctrl Pts',(19.1540296665579,-21.4788025811522,-20.8122573343165));
#51842=CARTESIAN_POINT('Ctrl Pts',(19.0678455531895,-21.4901385199818,-20.8165733748716));
#51843=CARTESIAN_POINT('Ctrl Pts',(18.9844645952716,-21.5011057551435,-20.8207490353481));
#51844=CARTESIAN_POINT('Ctrl Pts',(18.9006026815546,-21.5079520580807,-20.8249246958246));
#51845=CARTESIAN_POINT('Ctrl Pts',(18.816697839618,-21.5106639223084,-20.8291003563011));
#51846=CARTESIAN_POINT('Ctrl Pts',(18.7285618460937,-21.5135125403678,-20.8334865868954));
#51847=CARTESIAN_POINT('Ctrl Pts',(18.6403790644727,-21.511798786369,-20.8378728174898));
#51848=CARTESIAN_POINT('Ctrl Pts',(18.5526528282173,-21.5055687191236,-20.8422590480841));
#51849=CARTESIAN_POINT('Ctrl Pts',(18.4649265919619,-21.4993386518781,-20.8466452786785));
#51850=CARTESIAN_POINT('Ctrl Pts',(18.3776574674128,-21.4885924176826,-20.8510315092728));
#51851=CARTESIAN_POINT('Ctrl Pts',(18.2913357986938,-21.4734377654192,-20.8554177398671));
#51852=CARTESIAN_POINT('Ctrl Pts',(18.208977638002,-21.458978947548,-20.8596025742139));
#51853=CARTESIAN_POINT('Ctrl Pts',(18.1271754851468,-21.4404538825132,-20.8637874085605));
#51854=CARTESIAN_POINT('Ctrl Pts',(18.0463616913993,-21.4179184002202,-20.8679722429073));
#51855=CARTESIAN_POINT('Ctrl Pts',(17.9656628842856,-21.3954149827411,-20.8721511228247));
#51856=CARTESIAN_POINT('Ctrl Pts',(17.8859500822175,-21.3689126049628,-20.8763300027422));
#51857=CARTESIAN_POINT('Ctrl Pts',(17.8076468707951,-21.3385183594543,-20.8805088826597));
#51858=CARTESIAN_POINT('Ctrl Pts',(17.7279449213762,-21.3075811785374,-20.8847624103218));
#51859=CARTESIAN_POINT('Ctrl Pts',(17.6497038924681,-21.2726118027868,-20.8890159379838));
#51860=CARTESIAN_POINT('Ctrl Pts',(17.5733558319313,-21.2337767452422,-20.8932694656458));
#51861=CARTESIAN_POINT('Ctrl Pts',(17.4984833648361,-21.1956922602179,-20.8974407845723));
#51862=CARTESIAN_POINT('Ctrl Pts',(17.4254317742295,-21.1538904079626,-20.9016121034987));
#51863=CARTESIAN_POINT('Ctrl Pts',(17.3545880671759,-21.108576620383,-20.9057834224251));
#51864=CARTESIAN_POINT('Ctrl Pts',(17.2837681192032,-21.0632780298334,-20.909953342403));
#51865=CARTESIAN_POINT('Ctrl Pts',(17.2151549713756,-21.0144700907621,-20.9141232623808));
#51866=CARTESIAN_POINT('Ctrl Pts',(17.149108758861,-20.9624028834442,-20.9182931823587));
#51867=CARTESIAN_POINT('Ctrl Pts',(17.083064889567,-20.9103375233928,-20.922462954394));
#51868=CARTESIAN_POINT('Ctrl Pts',(17.0195881352145,-20.8550134104492,-20.9266327264293));
#51869=CARTESIAN_POINT('Ctrl Pts',(16.959006405508,-20.7967215886177,-20.9308024984647));
#51870=CARTESIAN_POINT('Ctrl Pts',(16.8963013133661,-20.7363866645942,-20.9351184191383));
#51871=CARTESIAN_POINT('Ctrl Pts',(16.8366983362716,-20.6728724968332,-20.939434339812));
#51872=CARTESIAN_POINT('Ctrl Pts',(16.780518958098,-20.6065427824416,-20.9437502604856));
#51873=CARTESIAN_POINT('Ctrl Pts',(16.7261638999388,-20.5423670012093,-20.9479260297243));
#51874=CARTESIAN_POINT('Ctrl Pts',(16.6750137422498,-20.4755561368783,-20.952101798963));
#51875=CARTESIAN_POINT('Ctrl Pts',(16.6273169433958,-20.4064712094149,-20.9562775682017));
#51876=CARTESIAN_POINT('Ctrl Pts',(16.5772188714759,-20.3339082335381,-20.9606635645928));
#51877=CARTESIAN_POINT('Ctrl Pts',(16.530931306338,-20.2588367080558,-20.965049560984));
#51878=CARTESIAN_POINT('Ctrl Pts',(16.4886879171311,-20.1817047005371,-20.9694355573751));
#51879=CARTESIAN_POINT('Ctrl Pts',(16.4464445279242,-20.1045726930183,-20.9738215537662));
#51880=CARTESIAN_POINT('Ctrl Pts',(16.408245498097,-20.0253807586023,-20.9782075501573));
#51881=CARTESIAN_POINT('Ctrl Pts',(16.374265613089,-19.9445994273774,-20.9825935465485));
#51882=CARTESIAN_POINT('Ctrl Pts',(16.3382155102257,-19.8588965093302,-20.9872467589128));
#51883=CARTESIAN_POINT('Ctrl Pts',(16.30679887472,-19.7711342279521,-20.9918999712772));
#51884=CARTESIAN_POINT('Ctrl Pts',(16.2802296059439,-19.6818019274115,-20.9965531836415));
#51885=CARTESIAN_POINT('Ctrl Pts',(16.2537435506638,-19.5927494107485,-21.0011918223993));
#51886=CARTESIAN_POINT('Ctrl Pts',(16.2320746955043,-19.5021369352023,-21.0058304611572));
#51887=CARTESIAN_POINT('Ctrl Pts',(16.2153886011344,-19.4104720509521,-21.010469099915));
#51888=CARTESIAN_POINT('Ctrl Pts',(16.1987928068799,-19.3193032294376,-21.0150826357574));
#51889=CARTESIAN_POINT('Ctrl Pts',(16.1871261077823,-19.2270936177058,-21.0196961715999));
#51890=CARTESIAN_POINT('Ctrl Pts',(16.1805035115345,-19.1343614087313,-21.0243097074423));
#51891=CARTESIAN_POINT('Ctrl Pts',(16.1762064899349,-19.0741928147187,-21.0273031653588));
#51892=CARTESIAN_POINT('Ctrl Pts',(16.1740320413834,-19.0138045835855,-21.0302966232753));
#51893=CARTESIAN_POINT('Ctrl Pts',(16.1740003516178,-18.9533417463077,-21.0332900811918));
#51894=CARTESIAN_POINT('Ctrl Pts',(16.1775161375017,-18.9533393271451,-21.0332901097715));
#51895=CARTESIAN_POINT('Ctrl Pts',(16.179969922226,-18.4391275102653,-21.0587831909243));
#51896=CARTESIAN_POINT('Ctrl Pts',(16.5801691895444,-17.06634175119,-21.1266682076376));
#51897=CARTESIAN_POINT('Ctrl Pts',(18.4990491880931,-16.0899931954376,-21.2211093027264));
#51898=CARTESIAN_POINT('Ctrl Pts',(19.8649654422083,-16.6008610266685,-21.2900573166623));
#51899=CARTESIAN_POINT('Ctrl Pts',(20.2916907304466,-16.9243022127157,-21.3166133950378));
#51900=CARTESIAN_POINT('',(16.1715628046961,-18.9501455684938,-20.9667098902285));
#51901=CARTESIAN_POINT('Ctrl Pts',(16.1715628046961,-18.9501455684938,-20.9667098902285));
#51902=CARTESIAN_POINT('Ctrl Pts',(16.1706210062014,-18.8345295298074,-20.9724759609646));
#51903=CARTESIAN_POINT('Ctrl Pts',(16.2303035994096,-17.8698877850362,-21.0206339672611));
#51904=CARTESIAN_POINT('Ctrl Pts',(17.4553333973082,-16.2082456258976,-21.1111839091181));
#51905=CARTESIAN_POINT('Ctrl Pts',(19.4740835894722,-16.3361983067415,-21.1999086076436));
#51906=CARTESIAN_POINT('Ctrl Pts',(20.2333094787133,-16.8707090063625,-21.2462413706087));
#51907=CARTESIAN_POINT('Ctrl Pts',(20.2955778924961,-16.9192440454753,-21.2501821980133));
#51908=CARTESIAN_POINT('Ctrl Pts',(20.2940725979671,-16.9211546778497,-20.4499991793503));
#51909=CARTESIAN_POINT('Ctrl Pts',(20.4294543463688,-17.0229918862778,-20.4584344114705));
#51910=CARTESIAN_POINT('Ctrl Pts',(21.1817798484721,-17.716545109861,-20.5092615791512));
#51911=CARTESIAN_POINT('Ctrl Pts',(21.6424139385631,-19.7912991649835,-20.6024806823924));
#51912=CARTESIAN_POINT('Ctrl Pts',(19.6025526266728,-21.851808827879,-20.7296564890738));
#51913=CARTESIAN_POINT('Ctrl Pts',(16.8944629917136,-21.2791319918735,-20.8510662250192));
#51914=CARTESIAN_POINT('Ctrl Pts',(16.1775450733739,-19.6845343053476,-20.9300840254041));
#51915=CARTESIAN_POINT('Ctrl Pts',(16.1715628046961,-18.9501455684938,-20.9667098902285));
#51916=CARTESIAN_POINT('Origin',(18.734,-18.952,1.76670989022851));
#51917=CARTESIAN_POINT('',(20.293535888361,-16.9218650751947,-19.6501081160065));
#51918=CARTESIAN_POINT('',(20.293535888361,-16.9218650751948,-19.716724552643));
#51919=CARTESIAN_POINT('',(20.293535888361,-16.9218650751948,1.76670989022851));
#51920=CARTESIAN_POINT('',(16.1740004726297,-18.9535555911146,-20.2332901098006));
#51921=CARTESIAN_POINT('Ctrl Pts',(20.293535888361,-16.9218650751948,-19.716724552643));
#51922=CARTESIAN_POINT('Ctrl Pts',(20.3599060643816,-16.9728501945365,-19.720906221147));
#51923=CARTESIAN_POINT('Ctrl Pts',(20.4238851560338,-17.0271793245034,-19.725087889651));
#51924=CARTESIAN_POINT('Ctrl Pts',(20.4851178704728,-17.0845990779399,-19.729269558155));
#51925=CARTESIAN_POINT('Ctrl Pts',(20.5462729423841,-17.1419460236487,-19.7334459243412));
#51926=CARTESIAN_POINT('Ctrl Pts',(20.6046882218323,-17.2023754951433,-19.7376222905273));
#51927=CARTESIAN_POINT('Ctrl Pts',(20.6600404295884,-17.2655930907427,-19.7417986567135));
#51928=CARTESIAN_POINT('Ctrl Pts',(20.7153403235321,-17.3287509388888,-19.7459710757827));
#51929=CARTESIAN_POINT('Ctrl Pts',(20.767582597195,-17.3946913295733,-19.7501434948519));
#51930=CARTESIAN_POINT('Ctrl Pts',(20.8164808501031,-17.4630831087821,-19.7543159139211));
#51931=CARTESIAN_POINT('Ctrl Pts',(20.8653546247269,-17.5314406513197,-19.7584862442928));
#51932=CARTESIAN_POINT('Ctrl Pts',(20.9108874353274,-17.6022467722473,-19.7626565746645));
#51933=CARTESIAN_POINT('Ctrl Pts',(20.9528339582812,-17.6751382746835,-19.7668269050362));
#51934=CARTESIAN_POINT('Ctrl Pts',(20.994772065989,-17.7480151537402,-19.7709963987627));
#51935=CARTESIAN_POINT('Ctrl Pts',(21.0331250860997,-17.8229761845117,-19.7751658924892));
#51936=CARTESIAN_POINT('Ctrl Pts',(21.0676924595754,-17.8996314789386,-19.7793353862157));
#51937=CARTESIAN_POINT('Ctrl Pts',(21.1022632674651,-17.9762943893915,-19.7835052941989));
#51938=CARTESIAN_POINT('Ctrl Pts',(21.1330474939752,-18.0546514778417,-19.7876752021822));
#51939=CARTESIAN_POINT('Ctrl Pts',(21.1598923176434,-18.134291945008,-19.7918451101654));
#51940=CARTESIAN_POINT('Ctrl Pts',(21.1867656122562,-18.21401687685,-19.7960194406482));
#51941=CARTESIAN_POINT('Ctrl Pts',(21.2096910150703,-18.2950274681917,-19.8001937711309));
#51942=CARTESIAN_POINT('Ctrl Pts',(21.2285654637021,-18.3768972723899,-19.8043681016137));
#51943=CARTESIAN_POINT('Ctrl Pts',(21.2474505170233,-18.4588130754865,-19.8085447774618));
#51944=CARTESIAN_POINT('Ctrl Pts',(21.2622800033412,-18.5415885996961,-19.8127214533099));
#51945=CARTESIAN_POINT('Ctrl Pts',(21.2730023687634,-18.624789102544,-19.816898129158));
#51946=CARTESIAN_POINT('Ctrl Pts',(21.2837431250598,-18.7081323099092,-19.821081968791));
#51947=CARTESIAN_POINT('Ctrl Pts',(21.290362656088,-18.7919014928153,-19.8252658084241));
#51948=CARTESIAN_POINT('Ctrl Pts',(21.2928614752057,-18.8756589841044,-19.8294496480571));
#51949=CARTESIAN_POINT('Ctrl Pts',(21.2945659689631,-18.9327916192854,-19.83230352751));
#51950=CARTESIAN_POINT('Ctrl Pts',(21.2943542420303,-18.9899188035593,-19.8351574069628));
#51951=CARTESIAN_POINT('Ctrl Pts',(21.2922402934573,-19.0469031133929,-19.8380112864157));
#51952=CARTESIAN_POINT('Ctrl Pts',(21.2891406189066,-19.1304589847303,-19.8421959187306));
#51953=CARTESIAN_POINT('Ctrl Pts',(21.2819372856921,-19.2140183312952,-19.8463805510455));
#51954=CARTESIAN_POINT('Ctrl Pts',(21.2706266468765,-19.2971452655857,-19.8505651833604));
#51955=CARTESIAN_POINT('Ctrl Pts',(21.2593321073624,-19.380153878921,-19.8547438593665));
#51956=CARTESIAN_POINT('Ctrl Pts',(21.243941936219,-19.4627308505955,-19.8589225353726));
#51957=CARTESIAN_POINT('Ctrl Pts',(21.2245044655718,-19.5444419861614,-19.8631012113787));
#51958=CARTESIAN_POINT('Ctrl Pts',(21.2047185799778,-19.6276177866251,-19.8673547897837));
#51959=CARTESIAN_POINT('Ctrl Pts',(21.1807388847111,-19.7098959225239,-19.8716083681886));
#51960=CARTESIAN_POINT('Ctrl Pts',(21.1526714444945,-19.7908256336015,-19.8758619465935));
#51961=CARTESIAN_POINT('Ctrl Pts',(21.125148163346,-19.8701863153761,-19.8800330585091));
#51962=CARTESIAN_POINT('Ctrl Pts',(21.0936943831976,-19.9482499363987,-19.8842041704246));
#51963=CARTESIAN_POINT('Ctrl Pts',(21.0584608475263,-20.0246051315918,-19.8883752823401));
#51964=CARTESIAN_POINT('Ctrl Pts',(21.0232391347282,-20.1009347052351,-19.8925449946083));
#51965=CARTESIAN_POINT('Ctrl Pts',(20.9842403779078,-20.1755565742226,-19.8967147068764));
#51966=CARTESIAN_POINT('Ctrl Pts',(20.9416632153647,-20.2480799078473,-19.9008844191445));
#51967=CARTESIAN_POINT('Ctrl Pts',(20.89908756777,-20.3206006610016,-19.9050539830491));
#51968=CARTESIAN_POINT('Ctrl Pts',(20.8529340012468,-20.3910226309664,-19.9092235469537));
#51969=CARTESIAN_POINT('Ctrl Pts',(20.8034461281557,-20.4589813279074,-19.9133931108583));
#51970=CARTESIAN_POINT('Ctrl Pts',(20.7522182683888,-20.5293294430996,-19.9177092760448));
#51971=CARTESIAN_POINT('Ctrl Pts',(20.6974175740299,-20.5970374130935,-19.9220254412314));
#51972=CARTESIAN_POINT('Ctrl Pts',(20.6393606095101,-20.6617370990089,-19.926341606418));
#51973=CARTESIAN_POINT('Ctrl Pts',(20.5831949030825,-20.7243291341788,-19.9305171686225));
#51974=CARTESIAN_POINT('Ctrl Pts',(20.523982186015,-20.784105569659,-19.9346927308271));
#51975=CARTESIAN_POINT('Ctrl Pts',(20.4620462261043,-20.8407710926543,-19.9388682930317));
#51976=CARTESIAN_POINT('Ctrl Pts',(20.396981927938,-20.900298748143,-19.9432547597093));
#51977=CARTESIAN_POINT('Ctrl Pts',(20.3289124964612,-20.9563925858392,-19.9476412263868));
#51978=CARTESIAN_POINT('Ctrl Pts',(20.2582501417943,-21.0087599532371,-19.9520276930644));
#51979=CARTESIAN_POINT('Ctrl Pts',(20.1875877871275,-21.061127320635,-19.9564141597419));
#51980=CARTESIAN_POINT('Ctrl Pts',(20.1143330347169,-21.1097679601497,-19.9608006264195));
#51981=CARTESIAN_POINT('Ctrl Pts',(20.0389283877474,-21.1544445288931,-19.965187093097));
#51982=CARTESIAN_POINT('Ctrl Pts',(19.9669932812531,-21.1970654264043,-19.9693717283982));
#51983=CARTESIAN_POINT('Ctrl Pts',(19.8928340180601,-21.2362376726233,-19.9735563636995));
#51984=CARTESIAN_POINT('Ctrl Pts',(19.8168151370649,-21.2717222633201,-19.9777409990007));
#51985=CARTESIAN_POINT('Ctrl Pts',(19.7409044598143,-21.3071563459651,-19.9819196779762));
#51986=CARTESIAN_POINT('Ctrl Pts',(19.6631398357117,-21.3389130062059,-19.9860983569518));
#51987=CARTESIAN_POINT('Ctrl Pts',(19.5839125153236,-21.3667978624093,-19.9902770359274));
#51988=CARTESIAN_POINT('Ctrl Pts',(19.5032651236309,-21.3951825270617,-19.9945306135879));
#51989=CARTESIAN_POINT('Ctrl Pts',(19.4211024978227,-21.4195549746049,-19.9987841912483));
#51990=CARTESIAN_POINT('Ctrl Pts',(19.3378610660991,-21.4397604010133,-20.0030377689088));
#51991=CARTESIAN_POINT('Ctrl Pts',(19.2562334111026,-21.4595741108662,-20.007208883732));
#51992=CARTESIAN_POINT('Ctrl Pts',(19.1735688735353,-21.4753808138571,-20.0113799985552));
#51993=CARTESIAN_POINT('Ctrl Pts',(19.0902949413619,-21.4870845971604,-20.0155511133785));
#51994=CARTESIAN_POINT('Ctrl Pts',(19.0070489529337,-21.4987844530938,-20.0197208285252));
#51995=CARTESIAN_POINT('Ctrl Pts',(18.9231944311979,-21.5063840596987,-20.0238905436719));
#51996=CARTESIAN_POINT('Ctrl Pts',(18.8391675225314,-21.509838890979,-20.0280602588185));
#51997=CARTESIAN_POINT('Ctrl Pts',(18.7551436043038,-21.513293599305,-20.032229825569));
#51998=CARTESIAN_POINT('Ctrl Pts',(18.670947771023,-21.5126038075443,-20.0363993923194));
#51999=CARTESIAN_POINT('Ctrl Pts',(18.5870183641846,-21.5077770635822,-20.0405689590698));
#52000=CARTESIAN_POINT('Ctrl Pts',(18.5001381401371,-21.5027806193961,-20.0448851207956));
#52001=CARTESIAN_POINT('Ctrl Pts',(18.4135439525319,-21.4933509339464,-20.0492012825213));
#52002=CARTESIAN_POINT('Ctrl Pts',(18.3277166966688,-21.4795549207553,-20.053517444247));
#52003=CARTESIAN_POINT('Ctrl Pts',(18.2446852202507,-21.4662083057154,-20.0576930091878));
#52004=CARTESIAN_POINT('Ctrl Pts',(18.1623719289166,-21.4487756010914,-20.0618685741286));
#52005=CARTESIAN_POINT('Ctrl Pts',(18.0812003839157,-21.4273691969563,-20.0660441390694));
#52006=CARTESIAN_POINT('Ctrl Pts',(17.9959291092672,-21.4048816199831,-20.0704305991875));
#52007=CARTESIAN_POINT('Ctrl Pts',(17.9119185059158,-21.3780085540391,-20.0748170593057));
#52008=CARTESIAN_POINT('Ctrl Pts',(17.8296377675495,-21.3469381938825,-20.0792035194239));
#52009=CARTESIAN_POINT('Ctrl Pts',(17.7473570291832,-21.315867833726,-20.0835899795421));
#52010=CARTESIAN_POINT('Ctrl Pts',(17.6668066567987,-21.2806004817434,-20.0879764396603));
#52011=CARTESIAN_POINT('Ctrl Pts',(17.5884257348681,-21.2413797419973,-20.0923628997785));
#52012=CARTESIAN_POINT('Ctrl Pts',(17.5136510990602,-21.2039635384314,-20.0965475399912));
#52013=CARTESIAN_POINT('Ctrl Pts',(17.4405723466444,-21.1628104733658,-20.100732180204));
#52014=CARTESIAN_POINT('Ctrl Pts',(17.3695877608619,-21.1180976990178,-20.1049168204167));
#52015=CARTESIAN_POINT('Ctrl Pts',(17.2987042121431,-21.0734485673238,-20.1090955043538));
#52016=CARTESIAN_POINT('Ctrl Pts',(17.2299092952355,-21.0252500336355,-20.1132741882909));
#52017=CARTESIAN_POINT('Ctrl Pts',(17.1635782312554,-20.9737258637741,-20.117452872228));
#52018=CARTESIAN_POINT('Ctrl Pts',(17.0960583483627,-20.9212782516533,-20.1217064486544));
#52019=CARTESIAN_POINT('Ctrl Pts',(17.0310919385808,-20.8653848344035,-20.1259600250807));
#52020=CARTESIAN_POINT('Ctrl Pts',(16.9690453966424,-20.8063287864041,-20.130213601507));
#52021=CARTESIAN_POINT('Ctrl Pts',(16.9082016411681,-20.748417553457,-20.1343847213775));
#52022=CARTESIAN_POINT('Ctrl Pts',(16.8501659076099,-20.6874655440672,-20.138555841248));
#52023=CARTESIAN_POINT('Ctrl Pts',(16.7952502349276,-20.6237802931102,-20.1427269611185));
#52024=CARTESIAN_POINT('Ctrl Pts',(16.7403529896792,-20.5601164122958,-20.1468966813333));
#52025=CARTESIAN_POINT('Ctrl Pts',(16.6885740261885,-20.4937214595179,-20.151066401548));
#52026=CARTESIAN_POINT('Ctrl Pts',(16.6401868618211,-20.4249380646821,-20.1552361217628));
#52027=CARTESIAN_POINT('Ctrl Pts',(16.5918014193429,-20.3561571175489,-20.1594056935953));
#52028=CARTESIAN_POINT('Ctrl Pts',(16.5468077999962,-20.2849882740964,-20.1635752654278));
#52029=CARTESIAN_POINT('Ctrl Pts',(16.5054369234077,-20.2118041965518,-20.1677448372603));
#52030=CARTESIAN_POINT('Ctrl Pts',(16.4626116274946,-20.136047286488,-20.1720609930269));
#52031=CARTESIAN_POINT('Ctrl Pts',(16.4236688015119,-20.0581312666225,-20.1763771487935));
#52032=CARTESIAN_POINT('Ctrl Pts',(16.3888124800457,-19.978496710297,-20.1806933045602));
#52033=CARTESIAN_POINT('Ctrl Pts',(16.3550914981633,-19.9014560095544,-20.1848688745654));
#52034=CARTESIAN_POINT('Ctrl Pts',(16.3251950198264,-19.8228074630063,-20.1890444445707));
#52035=CARTESIAN_POINT('Ctrl Pts',(16.2992578088289,-19.7429680540524,-20.193220014576));
#52036=CARTESIAN_POINT('Ctrl Pts',(16.2720106919199,-19.6590965186773,-20.1976064632233));
#52037=CARTESIAN_POINT('Ctrl Pts',(16.2491334314107,-19.5739112339791,-20.2019929118706));
#52038=CARTESIAN_POINT('Ctrl Pts',(16.2307217504163,-19.4879085791077,-20.2063793605179));
#52039=CARTESIAN_POINT('Ctrl Pts',(16.2123100694219,-19.4019059242363,-20.2107658091652));
#52040=CARTESIAN_POINT('Ctrl Pts',(16.1983639848637,-19.3150864841139,-20.2151522578125));
#52041=CARTESIAN_POINT('Ctrl Pts',(16.1889163328206,-19.2279513128369,-20.2195387064599));
#52042=CARTESIAN_POINT('Ctrl Pts',(16.1790436177049,-19.1368958083959,-20.2241225075637));
#52043=CARTESIAN_POINT('Ctrl Pts',(16.1740562221029,-19.0453011470167,-20.2287063086676));
#52044=CARTESIAN_POINT('Ctrl Pts',(16.17400047263,-18.9535555916975,-20.2332901097715));
#52045=CARTESIAN_POINT('Ctrl Pts',(16.1740004726297,-18.9535555911146,-20.2332901098006));
#52046=CARTESIAN_POINT('Ctrl Pts',(16.173950276098,-18.8709483454626,-20.2374173417138));
#52047=CARTESIAN_POINT('Ctrl Pts',(16.1779027082632,-18.7881812209217,-20.2415445736269));
#52048=CARTESIAN_POINT('Ctrl Pts',(16.1858778001745,-18.7056805838826,-20.24567180554));
#52049=CARTESIAN_POINT('Ctrl Pts',(16.1940130436929,-18.6215232123815,-20.2498819183568));
#52050=CARTESIAN_POINT('Ctrl Pts',(16.2063343518257,-18.5376436404924,-20.2540920311735));
#52051=CARTESIAN_POINT('Ctrl Pts',(16.2228070334153,-18.4544963471735,-20.2583021439902));
#52052=CARTESIAN_POINT('Ctrl Pts',(16.2389199317137,-18.3731650913156,-20.2624203028504));
#52053=CARTESIAN_POINT('Ctrl Pts',(16.2590046102178,-18.2925349422861,-20.2665384617107));
#52054=CARTESIAN_POINT('Ctrl Pts',(16.2829763019886,-18.2130258246822,-20.270656620571));
#52055=CARTESIAN_POINT('Ctrl Pts',(16.306937024594,-18.1335530895192,-20.27477289501));
#52056=CARTESIAN_POINT('Ctrl Pts',(16.3347810947711,-18.0552008202622,-20.2788891694489));
#52057=CARTESIAN_POINT('Ctrl Pts',(16.3663732871523,-17.9783759716349,-20.2830054438879));
#52058=CARTESIAN_POINT('Ctrl Pts',(16.3979610860963,-17.9015618068228,-20.2871211458883));
#52059=CARTESIAN_POINT('Ctrl Pts',(16.4332957915605,-17.8262750781318,-20.2912368478886));
#52060=CARTESIAN_POINT('Ctrl Pts',(16.4721937794553,-17.7529034147721,-20.2953525498889));
#52061=CARTESIAN_POINT('Ctrl Pts',(16.5126461134818,-17.6765998526872,-20.2996327134933));
#52062=CARTESIAN_POINT('Ctrl Pts',(16.5569522564909,-17.6023681227906,-20.3039128770976));
#52063=CARTESIAN_POINT('Ctrl Pts',(16.6048536565105,-17.5306148136394,-20.308193040702));
#52064=CARTESIAN_POINT('Ctrl Pts',(16.6509736167644,-17.4615299901315,-20.3123140262104));
#52065=CARTESIAN_POINT('Ctrl Pts',(16.7004258077716,-17.3947428571309,-20.3164350117188));
#52066=CARTESIAN_POINT('Ctrl Pts',(16.752937145384,-17.3305839626854,-20.3205559972272));
#52067=CARTESIAN_POINT('Ctrl Pts',(16.8054841274566,-17.2663815174707,-20.3246797800421));
#52068=CARTESIAN_POINT('Ctrl Pts',(16.8610940674614,-17.2048112072835,-20.3288035628569));
#52069=CARTESIAN_POINT('Ctrl Pts',(16.9194565997149,-17.1461671593191,-20.3329273456718));
#52070=CARTESIAN_POINT('Ctrl Pts',(16.9779086863938,-17.0874331249574,-20.3370574562278));
#52071=CARTESIAN_POINT('Ctrl Pts',(17.0391214358428,-17.0316346193019,-20.3411875667839));
#52072=CARTESIAN_POINT('Ctrl Pts',(17.1027516837168,-16.9790253598631,-20.34531767734));
#52073=CARTESIAN_POINT('Ctrl Pts',(17.1099251001079,-16.9730944050642,-20.3457832892737));
#52074=CARTESIAN_POINT('Ctrl Pts',(17.117129212341,-16.9672039375623,-20.3462489012075));
#52075=CARTESIAN_POINT('Ctrl Pts',(17.1243635072392,-16.9613542853705,-20.3467145131413));
#52076=CARTESIAN_POINT('Ctrl Pts',(17.1893810782662,-16.9087810654215,-20.3508991582797));
#52077=CARTESIAN_POINT('Ctrl Pts',(17.2570980357154,-16.8592987213468,-20.3550838034181));
#52078=CARTESIAN_POINT('Ctrl Pts',(17.3271882231892,-16.8131964502025,-20.3592684485566));
#52079=CARTESIAN_POINT('Ctrl Pts',(17.3971786444276,-16.7671598009406,-20.3634471372793));
#52080=CARTESIAN_POINT('Ctrl Pts',(17.4695352047632,-16.7244939187135,-20.367625826002));
#52081=CARTESIAN_POINT('Ctrl Pts',(17.5438988654958,-16.6854477085997,-20.3718045147248));
#52082=CARTESIAN_POINT('Ctrl Pts',(17.6195952011134,-16.6457017494008,-20.3760580899372));
#52083=CARTESIAN_POINT('Ctrl Pts',(17.6973709112956,-16.6097067832357,-20.3803116651496));
#52084=CARTESIAN_POINT('Ctrl Pts',(17.7768165359456,-16.5776790831607,-20.384565240362));
#52085=CARTESIAN_POINT('Ctrl Pts',(17.8547221935641,-16.5462722052193,-20.388736364645));
#52086=CARTESIAN_POINT('Ctrl Pts',(17.9342331580126,-16.5186803432953,-20.392907488928));
#52087=CARTESIAN_POINT('Ctrl Pts',(18.0149402978771,-16.4950602073346,-20.3970786132109));
#52088=CARTESIAN_POINT('Ctrl Pts',(18.0956203529298,-16.4714479981438,-20.4012483376907));
#52089=CARTESIAN_POINT('Ctrl Pts',(18.1774953450108,-16.4518049968894,-20.4054180621704));
#52090=CARTESIAN_POINT('Ctrl Pts',(18.2601401459595,-16.4362383183758,-20.4095877866501));
#52091=CARTESIAN_POINT('Ctrl Pts',(18.3427820029266,-16.42067219438,-20.4137573625955));
#52092=CARTESIAN_POINT('Ctrl Pts',(18.4261931620005,-16.4091821887308,-20.4179269385409));
#52093=CARTESIAN_POINT('Ctrl Pts',(18.5099387943012,-16.401824206824,-20.4220965144863));
#52094=CARTESIAN_POINT('Ctrl Pts',(18.5966283648554,-16.3942075673155,-20.426412664931));
#52095=CARTESIAN_POINT('Ctrl Pts',(18.683675837258,-16.3910189213194,-20.4307288153757));
#52096=CARTESIAN_POINT('Ctrl Pts',(18.7705956997936,-16.3922615847012,-20.4350449658204));
#52097=CARTESIAN_POINT('Ctrl Pts',(18.8546845879849,-16.3934637746163,-20.4392205395221));
#52098=CARTESIAN_POINT('Ctrl Pts',(18.9386535841084,-16.3988129731103,-20.4433961132239));
#52099=CARTESIAN_POINT('Ctrl Pts',(19.0220673264253,-16.4082592082828,-20.4475716869256));
#52100=CARTESIAN_POINT('Ctrl Pts',(19.1096934356116,-16.4181824752605,-20.4519581257418));
#52101=CARTESIAN_POINT('Ctrl Pts',(19.1967061584436,-16.432627374484,-20.456344564558));
#52102=CARTESIAN_POINT('Ctrl Pts',(19.2826140303201,-16.4514755258674,-20.4607310033742));
#52103=CARTESIAN_POINT('Ctrl Pts',(19.3685219021966,-16.4703236772509,-20.4651174421904));
#52104=CARTESIAN_POINT('Ctrl Pts',(19.4533243836861,-16.4935748540295,-20.4695038810066));
#52105=CARTESIAN_POINT('Ctrl Pts',(19.5365517912807,-16.5210514973961,-20.4738903198228));
#52106=CARTESIAN_POINT('Ctrl Pts',(19.6159350029072,-16.5472590203528,-20.4780741531404));
#52107=CARTESIAN_POINT('Ctrl Pts',(19.6941808259681,-16.57740780265,-20.482257986458));
#52108=CARTESIAN_POINT('Ctrl Pts',(19.7708697962533,-16.6113802048138,-20.4864418197756));
#52109=CARTESIAN_POINT('Ctrl Pts',(19.8474630716383,-16.6453102151496,-20.4906204323749));
#52110=CARTESIAN_POINT('Ctrl Pts',(19.9225029327703,-16.6830541923724,-20.4947990449742));
#52111=CARTESIAN_POINT('Ctrl Pts',(19.9955857717825,-16.7244449859911,-20.4989776575735));
#52112=CARTESIAN_POINT('Ctrl Pts',(20.0685856282316,-16.7657887820631,-20.5031515255298));
#52113=CARTESIAN_POINT('Ctrl Pts',(20.1396324806856,-16.8107709395873,-20.507325393486));
#52114=CARTESIAN_POINT('Ctrl Pts',(20.2083448692775,-16.859177215712,-20.5114992614423));
#52115=CARTESIAN_POINT('Ctrl Pts',(20.2371610874347,-16.8794775697176,-20.5132496748983));
#52116=CARTESIAN_POINT('Ctrl Pts',(20.2655670197412,-16.9003795799026,-20.5150000883544));
#52117=CARTESIAN_POINT('Ctrl Pts',(20.293535888361,-16.9218650751948,-20.5167505018104));
#52118=CARTESIAN_POINT('',(16.1742339566945,-18.9509923323772,-20.1667099326003));
#52119=CARTESIAN_POINT('Ctrl Pts',(16.1778405451444,-18.9509805605723,-20.166710586341));
#52120=CARTESIAN_POINT('Ctrl Pts',(16.17655678384,-18.5861666074448,-20.1847914783433));
#52121=CARTESIAN_POINT('Ctrl Pts',(16.4202751438729,-17.3676607662538,-20.2452643059062));
#52122=CARTESIAN_POINT('Ctrl Pts',(18.1401763667744,-16.0727553476898,-20.3396938369093));
#52123=CARTESIAN_POINT('Ctrl Pts',(19.749082511602,-16.5112008275589,-20.41604247591));
#52124=CARTESIAN_POINT('Ctrl Pts',(20.2940725979671,-16.9211546778497,-20.4499991793503));
#52125=CARTESIAN_POINT('Ctrl Pts',(20.293535888361,-16.9218650751947,-19.6501081160065));
#52126=CARTESIAN_POINT('Ctrl Pts',(20.3602263211758,-16.973096213635,-19.6542777831496));
#52127=CARTESIAN_POINT('Ctrl Pts',(20.4243867046238,-17.0276147056197,-19.6584474502926));
#52128=CARTESIAN_POINT('Ctrl Pts',(20.4856865660341,-17.0851325236172,-19.6626171174357));
#52129=CARTESIAN_POINT('Ctrl Pts',(20.5470483483268,-17.1427084421384,-19.6667909964883));
#52130=CARTESIAN_POINT('Ctrl Pts',(20.6055435003501,-17.2032894232085,-19.6709648755409));
#52131=CARTESIAN_POINT('Ctrl Pts',(20.6608777171633,-17.2665498336944,-19.6751387545935));
#52132=CARTESIAN_POINT('Ctrl Pts',(20.7162388992875,-17.3298410720612,-19.6793146676488));
#52133=CARTESIAN_POINT('Ctrl Pts',(20.7684357919223,-17.3958139797163,-19.6834905807041));
#52134=CARTESIAN_POINT('Ctrl Pts',(20.817215346003,-17.4641109509854,-19.6876664937594));
#52135=CARTESIAN_POINT('Ctrl Pts',(20.8660828502715,-17.5325310626062,-19.6918499360417));
#52136=CARTESIAN_POINT('Ctrl Pts',(20.9115204546417,-17.6032832230595,-19.696033378324));
#52137=CARTESIAN_POINT('Ctrl Pts',(20.9533193413648,-17.6759821078668,-19.7002168206063));
#52138=CARTESIAN_POINT('Ctrl Pts',(20.9933959861807,-17.745685576388,-19.7042278922783));
#52139=CARTESIAN_POINT('Ctrl Pts',(21.0301277554738,-17.8171781553883,-19.7082389639503));
#52140=CARTESIAN_POINT('Ctrl Pts',(21.0633723464495,-17.8901033611523,-19.7122500356223));
#52141=CARTESIAN_POINT('Ctrl Pts',(21.0980554588832,-17.9661841020042,-19.7164346697446));
#52142=CARTESIAN_POINT('Ctrl Pts',(21.1290718315276,-18.0441074153776,-19.7206193038669));
#52143=CARTESIAN_POINT('Ctrl Pts',(21.1562228177885,-18.1234852922339,-19.7248039379892));
#52144=CARTESIAN_POINT('Ctrl Pts',(21.1833351579802,-18.2027501845047,-19.7289826158026));
#52145=CARTESIAN_POINT('Ctrl Pts',(21.2065928926805,-18.2834650962588,-19.733161293616));
#52146=CARTESIAN_POINT('Ctrl Pts',(21.2258445987289,-18.3652202322969,-19.7373399714295));
#52147=CARTESIAN_POINT('Ctrl Pts',(21.2454413793526,-18.4484407771033,-19.7415935493826));
#52148=CARTESIAN_POINT('Ctrl Pts',(21.2608869019323,-18.5327387665071,-19.7458471273357));
#52149=CARTESIAN_POINT('Ctrl Pts',(21.2720739254928,-18.6176637190888,-19.7501007052888));
#52150=CARTESIAN_POINT('Ctrl Pts',(21.2830440658925,-18.7009422290717,-19.7542718189987));
#52151=CARTESIAN_POINT('Ctrl Pts',(21.2899192902196,-18.7848231321654,-19.7584429327087));
#52152=CARTESIAN_POINT('Ctrl Pts',(21.2926499549078,-18.8688711346757,-19.7626140464186));
#52153=CARTESIAN_POINT('Ctrl Pts',(21.2953797032961,-18.9528909340954,-19.7667837604725));
#52154=CARTESIAN_POINT('Ctrl Pts',(21.2939676391625,-19.0370772621645,-19.7709534745263));
#52155=CARTESIAN_POINT('Ctrl Pts',(21.2884161370488,-19.1209917121782,-19.7751231885802));
#52156=CARTESIAN_POINT('Ctrl Pts',(21.2828648324788,-19.2049031761925,-19.7792927542596));
#52157=CARTESIAN_POINT('Ctrl Pts',(21.2731744140114,-19.2885423224134,-19.783462319939));
#52158=CARTESIAN_POINT('Ctrl Pts',(21.2593992661682,-19.3714741308316,-19.7876318856184));
#52159=CARTESIAN_POINT('Ctrl Pts',(21.2451397991641,-19.4573217311042,-19.7919480486755));
#52160=CARTESIAN_POINT('Ctrl Pts',(21.2265031054957,-19.5424108076161,-19.7962642117326));
#52161=CARTESIAN_POINT('Ctrl Pts',(21.2036071461083,-19.6262703789215,-19.8005803747897));
#52162=CARTESIAN_POINT('Ctrl Pts',(21.1814570231881,-19.7073982225299,-19.804755938724));
#52163=CARTESIAN_POINT('Ctrl Pts',(21.1553210566129,-19.7873750003197,-19.8089315026582));
#52164=CARTESIAN_POINT('Ctrl Pts',(21.1253562910769,-19.8657916004906,-19.8131070665925));
#52165=CARTESIAN_POINT('Ctrl Pts',(21.0938780701788,-19.9481688531772,-19.817493529211));
#52166=CARTESIAN_POINT('Ctrl Pts',(21.0581743348026,-20.0288236424593,-19.8218799918296));
#52167=CARTESIAN_POINT('Ctrl Pts',(21.0184823804606,-20.1073095919991,-19.8262664544481));
#52168=CARTESIAN_POINT('Ctrl Pts',(20.9787904261185,-20.1857955415389,-19.8306529170666));
#52169=CARTESIAN_POINT('Ctrl Pts',(20.9351106070456,-20.262112185551,-19.8350393796852));
#52170=CARTESIAN_POINT('Ctrl Pts',(20.887732090269,-20.3358490103134,-19.8394258423037));
#52171=CARTESIAN_POINT('Ctrl Pts',(20.8425335350788,-20.4061930854412,-19.8436104767381));
#52172=CARTESIAN_POINT('Ctrl Pts',(20.7938009308873,-20.4744513619087,-19.8477951111725));
#52173=CARTESIAN_POINT('Ctrl Pts',(20.7417530082945,-20.5402467873993,-19.8519797456069));
#52174=CARTESIAN_POINT('Ctrl Pts',(20.6897791695075,-20.6059485612075,-19.8561584237297));
#52175=CARTESIAN_POINT('Ctrl Pts',(20.6344996686009,-20.669194089486,-19.8603371018525));
#52176=CARTESIAN_POINT('Ctrl Pts',(20.5761771160362,-20.729634234918,-19.8645157799753));
#52177=CARTESIAN_POINT('Ctrl Pts',(20.5168091743247,-20.7911577258021,-19.8687693578507));
#52178=CARTESIAN_POINT('Ctrl Pts',(20.4542882752172,-20.849773866077,-19.8730229357261));
#52179=CARTESIAN_POINT('Ctrl Pts',(20.3889351547385,-20.9051486460612,-19.8772765136015));
#52180=CARTESIAN_POINT('Ctrl Pts',(20.3248490313748,-20.9594498784325,-19.8814476276121));
#52181=CARTESIAN_POINT('Ctrl Pts',(20.2580398900243,-21.0106339980016,-19.8856187416226));
#52182=CARTESIAN_POINT('Ctrl Pts',(20.1888468727078,-21.0584236461292,-19.8897898556332));
#52183=CARTESIAN_POINT('Ctrl Pts',(20.119677073816,-21.1061972579516,-19.8939595699837));
#52184=CARTESIAN_POINT('Ctrl Pts',(20.0481253658498,-21.1505783992841,-19.8981292843343));
#52185=CARTESIAN_POINT('Ctrl Pts',(19.9745616647957,-21.1913317654692,-19.9022989986849));
#52186=CARTESIAN_POINT('Ctrl Pts',(19.9010005814965,-21.232083681451,-19.9064685646567));
#52187=CARTESIAN_POINT('Ctrl Pts',(19.8254280502834,-21.2692078567734,-19.9106381306285));
#52188=CARTESIAN_POINT('Ctrl Pts',(19.748239291486,-21.3025145520941,-19.9148076966003));
#52189=CARTESIAN_POINT('Ctrl Pts',(19.6683366724282,-21.3369922691832,-19.9191238592991));
#52190=CARTESIAN_POINT('Ctrl Pts',(19.5867025423585,-21.3673788575717,-19.9234400219978));
#52191=CARTESIAN_POINT('Ctrl Pts',(19.5037967719923,-21.3935185704455,-19.9277561846965));
#52192=CARTESIAN_POINT('Ctrl Pts',(19.423591647215,-21.4188067852878,-19.9319317489098));
#52193=CARTESIAN_POINT('Ctrl Pts',(19.3421969248401,-21.4401204858129,-19.936107313123));
#52194=CARTESIAN_POINT('Ctrl Pts',(19.2600416085035,-21.4573702772491,-19.9402828773363));
#52195=CARTESIAN_POINT('Ctrl Pts',(19.1737368242881,-21.4754913142561,-19.9446693392777));
#52196=CARTESIAN_POINT('Ctrl Pts',(19.0865931685419,-21.4891270269191,-19.9490558012192));
#52197=CARTESIAN_POINT('Ctrl Pts',(18.9991144164072,-21.4982353281292,-19.9534422631607));
#52198=CARTESIAN_POINT('Ctrl Pts',(18.9116356642725,-21.5073436293392,-19.9578287251022));
#52199=CARTESIAN_POINT('Ctrl Pts',(18.823822399141,-21.5119245648308,-19.9622151870437));
#52200=CARTESIAN_POINT('Ctrl Pts',(18.7361763184532,-21.5119990749291,-19.9666016489852));
#52201=CARTESIAN_POINT('Ctrl Pts',(18.6525629441398,-21.5120701567241,-19.9707862842974));
#52202=CARTESIAN_POINT('Ctrl Pts',(18.56879048318,-21.5080406575016,-19.9749709196097));
#52203=CARTESIAN_POINT('Ctrl Pts',(18.4852943717973,-21.4998904039421,-19.9791555549219));
#52204=CARTESIAN_POINT('Ctrl Pts',(18.401917106683,-21.4917517512489,-19.9833342339293));
#52205=CARTESIAN_POINT('Ctrl Pts',(18.3188158637713,-21.479504039016,-19.9875129129367));
#52206=CARTESIAN_POINT('Ctrl Pts',(18.2364263585066,-21.4631790998037,-19.9916915919441));
#52207=CARTESIAN_POINT('Ctrl Pts',(18.1525601036476,-21.4465615523608,-19.9959451695992));
#52208=CARTESIAN_POINT('Ctrl Pts',(18.0694318349348,-21.4257191735617,-20.0001987472543));
#52209=CARTESIAN_POINT('Ctrl Pts',(17.9874960097629,-21.4007408585965,-20.0044523249094));
#52210=CARTESIAN_POINT('Ctrl Pts',(17.9071486482338,-21.3762467902365,-20.0086234398147));
#52211=CARTESIAN_POINT('Ctrl Pts',(17.8279483680941,-21.3477758591386,-20.0127945547199));
#52212=CARTESIAN_POINT('Ctrl Pts',(17.750311955338,-21.3154631012117,-20.0169656696251));
#52213=CARTESIAN_POINT('Ctrl Pts',(17.6727015942353,-21.283161186145,-20.0211353848722));
#52214=CARTESIAN_POINT('Ctrl Pts',(17.5966544826743,-21.2470201811681,-20.0253051001192));
#52215=CARTESIAN_POINT('Ctrl Pts',(17.5225687032624,-21.2072237612451,-20.0294748153663));
#52216=CARTESIAN_POINT('Ctrl Pts',(17.4484855601721,-21.1674287574665,-20.0336443822352));
#52217=CARTESIAN_POINT('Ctrl Pts',(17.3763640153245,-21.1239788158134,-20.0378139491041));
#52218=CARTESIAN_POINT('Ctrl Pts',(17.3065775348649,-21.0771035518364,-20.041983515973));
#52219=CARTESIAN_POINT('Ctrl Pts',(17.2343374822407,-21.0285802345094,-20.0462996776141));
#52220=CARTESIAN_POINT('Ctrl Pts',(17.1646001862986,-20.9763865421865,-20.0506158392553));
#52221=CARTESIAN_POINT('Ctrl Pts',(17.0977455243703,-20.920824850255,-20.0549320008964));
#52222=CARTESIAN_POINT('Ctrl Pts',(17.0330686154625,-20.8670730491964,-20.059107565999));
#52223=CARTESIAN_POINT('Ctrl Pts',(16.9710897386263,-20.810169654399,-20.0632831311016));
#52224=CARTESIAN_POINT('Ctrl Pts',(16.9121162723823,-20.7504270024224,-20.0674586962043));
#52225=CARTESIAN_POINT('Ctrl Pts',(16.8501642397595,-20.6876669348876,-20.0718451561147));
#52226=CARTESIAN_POINT('Ctrl Pts',(16.7915295867437,-20.6217736911657,-20.0762316160251));
#52227=CARTESIAN_POINT('Ctrl Pts',(16.7365203854165,-20.5531480847578,-20.0806180759355));
#52228=CARTESIAN_POINT('Ctrl Pts',(16.6815111840894,-20.4845224783498,-20.0850045358459));
#52229=CARTESIAN_POINT('Ctrl Pts',(16.6301277117734,-20.4131650245491,-20.0893909957563));
#52230=CARTESIAN_POINT('Ctrl Pts',(16.5826239199876,-20.339508905323,-20.0937774556667));
#52231=CARTESIAN_POINT('Ctrl Pts',(16.5362791661252,-20.2676499107529,-20.0980568909966));
#52232=CARTESIAN_POINT('Ctrl Pts',(16.4934601213991,-20.1933453656254,-20.1023363263266));
#52233=CARTESIAN_POINT('Ctrl Pts',(16.4544271376053,-20.1169667656347,-20.1066157616565));
#52234=CARTESIAN_POINT('Ctrl Pts',(16.4154575008855,-20.0407121213442,-20.1108882518421));
#52235=CARTESIAN_POINT('Ctrl Pts',(16.3802619051423,-19.9623904954392,-20.1151607420277));
#52236=CARTESIAN_POINT('Ctrl Pts',(16.3490570393213,-19.882401566158,-20.1194332322133));
#52237=CARTESIAN_POINT('Ctrl Pts',(16.3179055660145,-19.8025495004692,-20.1236984120328));
#52238=CARTESIAN_POINT('Ctrl Pts',(16.2907313869642,-19.7210362103122,-20.1279635918524));
#52239=CARTESIAN_POINT('Ctrl Pts',(16.2677042874668,-19.6382838030585,-20.1322287716719));
#52240=CARTESIAN_POINT('Ctrl Pts',(16.2447004012897,-19.5556148174328,-20.136489651819));
#52241=CARTESIAN_POINT('Ctrl Pts',(16.2258353999309,-19.4717096122622,-20.1407505319661));
#52242=CARTESIAN_POINT('Ctrl Pts',(16.2112300227482,-19.3870076342743,-20.1450114121132));
#52243=CARTESIAN_POINT('Ctrl Pts',(16.1966372356338,-19.3023786707434,-20.1492686193135));
#52244=CARTESIAN_POINT('Ctrl Pts',(16.1862968405519,-19.2169547258213,-20.1535258265139));
#52245=CARTESIAN_POINT('Ctrl Pts',(16.1802787590759,-19.1311865610278,-20.1577830337143));
#52246=CARTESIAN_POINT('Ctrl Pts',(16.1760723590192,-19.0712380185088,-20.1607586525524));
#52247=CARTESIAN_POINT('Ctrl Pts',(16.1739765481552,-19.0111215762638,-20.1637342713904));
#52248=CARTESIAN_POINT('Ctrl Pts',(16.1740001980189,-18.950993095359,-20.1667098902285));
#52249=CARTESIAN_POINT('Origin',(18.734,-18.952,1.76670989022851));
#52250=CARTESIAN_POINT('',(20.293535888361,-16.9218650751948,-18.8501886412182));
#52251=CARTESIAN_POINT('',(20.2933494025377,-16.9221164381228,-18.9165759009586));
#52252=CARTESIAN_POINT('',(20.293535888361,-16.9218650751948,1.76670989022851));
#52253=CARTESIAN_POINT('',(16.1740009418753,-18.9498040034616,-19.4332901097715));
#52254=CARTESIAN_POINT('Ctrl Pts',(20.2933494025375,-16.9221164381226,-18.9165759009586));
#52255=CARTESIAN_POINT('Ctrl Pts',(20.460481259063,-17.0478571352914,-18.9269774805209));
#52256=CARTESIAN_POINT('Ctrl Pts',(21.2286611541766,-17.7870025066956,-18.9797709956437));
#52257=CARTESIAN_POINT('Ctrl Pts',(21.6004478622574,-19.9250196443109,-19.074956446327));
#52258=CARTESIAN_POINT('Ctrl Pts',(19.4673983198524,-21.8889061091152,-19.2021322530084));
#52259=CARTESIAN_POINT('Ctrl Pts',(16.8320816481898,-21.2027757351818,-19.3215765971073));
#52260=CARTESIAN_POINT('Ctrl Pts',(16.1790132429278,-19.6455867561426,-19.3986290056455));
#52261=CARTESIAN_POINT('Ctrl Pts',(16.1726852643248,-18.9498155443718,-19.4332894786233));
#52262=CARTESIAN_POINT('Ctrl Pts',(16.1740009418753,-18.9498040034616,-19.4332901097715));
#52263=CARTESIAN_POINT('Ctrl Pts',(16.1741094126172,-18.8233534412475,-19.4395926510339));
#52264=CARTESIAN_POINT('Ctrl Pts',(16.1835900621658,-18.6972910723228,-19.4458951922963));
#52265=CARTESIAN_POINT('Ctrl Pts',(16.2022529884095,-18.572715055265,-19.4521977335588));
#52266=CARTESIAN_POINT('Ctrl Pts',(16.2064836512073,-18.5444751579424,-19.4536264444963));
#52267=CARTESIAN_POINT('Ctrl Pts',(16.2111860003678,-18.5163115073012,-19.4550551554338));
#52268=CARTESIAN_POINT('Ctrl Pts',(16.2163575306343,-18.4882367021355,-19.4564838663713));
#52269=CARTESIAN_POINT('Ctrl Pts',(16.2315047248245,-18.4060067810516,-19.4606685004925));
#52270=CARTESIAN_POINT('Ctrl Pts',(16.25071296974,-18.3243667083971,-19.4648531346137));
#52271=CARTESIAN_POINT('Ctrl Pts',(16.2739228554016,-18.2437483197165,-19.469037768735));
#52272=CARTESIAN_POINT('Ctrl Pts',(16.2970997046629,-18.1632446813365,-19.4732164465473));
#52273=CARTESIAN_POINT('Ctrl Pts',(16.3242667547544,-18.0837602766464,-19.4773951243597));
#52274=CARTESIAN_POINT('Ctrl Pts',(16.3553134075097,-18.0057177510347,-19.4815738021721));
#52275=CARTESIAN_POINT('Ctrl Pts',(16.3869165517615,-17.9262763628078,-19.4858273801254));
#52276=CARTESIAN_POINT('Ctrl Pts',(16.4225396637624,-17.8483295278622,-19.4900809580788));
#52277=CARTESIAN_POINT('Ctrl Pts',(16.4620126245779,-17.7723079359755,-19.4943345360321));
#52278=CARTESIAN_POINT('Ctrl Pts',(16.5007203219077,-17.6977601769908,-19.498505649741));
#52279=CARTESIAN_POINT('Ctrl Pts',(16.5431297041304,-17.6250641048156,-19.5026767634499));
#52280=CARTESIAN_POINT('Ctrl Pts',(16.5890321382659,-17.5546049691916,-19.5068478771588));
#52281=CARTESIAN_POINT('Ctrl Pts',(16.634919169412,-17.484169476787,-19.5110175912116));
#52282=CARTESIAN_POINT('Ctrl Pts',(16.6842966737064,-17.4159698153114,-19.5151873052644));
#52283=CARTESIAN_POINT('Ctrl Pts',(16.7369115952916,-17.3503639914827,-19.5193570193173));
#52284=CARTESIAN_POINT('Ctrl Pts',(16.7895246446353,-17.2847605021618,-19.5235265849956));
#52285=CARTESIAN_POINT('Ctrl Pts',(16.8453745937438,-17.2217510253186,-19.527696150674));
#52286=CARTESIAN_POINT('Ctrl Pts',(16.9041676934287,-17.1616610014224,-19.5318657163523));
#52287=CARTESIAN_POINT('Ctrl Pts',(16.9650278943521,-17.0994582778473,-19.5361818794107));
#52288=CARTESIAN_POINT('Ctrl Pts',(17.0290416909462,-17.0403845007301,-19.540498042469));
#52289=CARTESIAN_POINT('Ctrl Pts',(17.0958426218327,-16.984758173392,-19.5448142055274));
#52290=CARTESIAN_POINT('Ctrl Pts',(17.1604675106391,-16.9309438751296,-19.5489897694607));
#52291=CARTESIAN_POINT('Ctrl Pts',(17.2277003349621,-16.8803561190544,-19.5531653333939));
#52292=CARTESIAN_POINT('Ctrl Pts',(17.2971780335747,-16.8332403069725,-19.5573408973272));
#52293=CARTESIAN_POINT('Ctrl Pts',(17.370164900217,-16.7837447773015,-19.5617273599481));
#52294=CARTESIAN_POINT('Ctrl Pts',(17.4456288796107,-16.7380814487272,-19.5661138225691));
#52295=CARTESIAN_POINT('Ctrl Pts',(17.523119783767,-16.696480303359,-19.57050028519));
#52296=CARTESIAN_POINT('Ctrl Pts',(17.6006106879233,-16.6548791579908,-19.5748867478109));
#52297=CARTESIAN_POINT('Ctrl Pts',(17.6801279596806,-16.6173403747401,-19.5792732104318));
#52298=CARTESIAN_POINT('Ctrl Pts',(17.7611994326909,-16.5840348279075,-19.5836596730528));
#52299=CARTESIAN_POINT('Ctrl Pts',(17.8385406770861,-16.5522617227492,-19.587844307487));
#52300=CARTESIAN_POINT('Ctrl Pts',(17.9175841221718,-16.5242225928453,-19.5920289419213));
#52301=CARTESIAN_POINT('Ctrl Pts',(17.9979345050501,-16.5001012282021,-19.5962135763556));
#52302=CARTESIAN_POINT('Ctrl Pts',(18.078170519057,-16.4760141973499,-19.6003922544782));
#52303=CARTESIAN_POINT('Ctrl Pts',(18.1597093389465,-16.4558339863015,-19.6045709326009));
#52304=CARTESIAN_POINT('Ctrl Pts',(18.2421357220942,-16.4396963694409,-19.6087496107236));
#52305=CARTESIAN_POINT('Ctrl Pts',(18.3260395379465,-16.4232694975869,-19.613003188599));
#52306=CARTESIAN_POINT('Ctrl Pts',(18.4108626031779,-16.411031755533,-19.6172567664745));
#52307=CARTESIAN_POINT('Ctrl Pts',(18.4961506937665,-16.4030732243699,-19.6215103443499));
#52308=CARTESIAN_POINT('Ctrl Pts',(18.5797853091396,-16.3952689847841,-19.6256814583603));
#52309=CARTESIAN_POINT('Ctrl Pts',(18.6638666007976,-16.3915795598322,-19.6298525723707));
#52310=CARTESIAN_POINT('Ctrl Pts',(18.7479577055537,-16.3920380505844,-19.634023686381));
#52311=CARTESIAN_POINT('Ctrl Pts',(18.8320205926793,-16.3924963874854,-19.6381934007314));
#52312=CARTESIAN_POINT('Ctrl Pts',(18.9160928267199,-16.3970998732974,-19.6423631150818));
#52313=CARTESIAN_POINT('Ctrl Pts',(18.9997364062972,-16.4058295103493,-19.6465328294322));
#52314=CARTESIAN_POINT('Ctrl Pts',(19.0833770094284,-16.4145588367581,-19.6507023954039));
#52315=CARTESIAN_POINT('Ctrl Pts',(19.1665885309651,-16.4274139738732,-19.6548719613755));
#52316=CARTESIAN_POINT('Ctrl Pts',(19.2489383260598,-16.444324079879,-19.6590415273471));
#52317=CARTESIAN_POINT('Ctrl Pts',(19.3341834370064,-16.461828724073,-19.6633576900461));
#52318=CARTESIAN_POINT('Ctrl Pts',(19.4185045808358,-16.4836786817424,-19.667673852745));
#52319=CARTESIAN_POINT('Ctrl Pts',(19.5014355882166,-16.5097382167469,-19.6719900154439));
#52320=CARTESIAN_POINT('Ctrl Pts',(19.5816651279086,-16.5349488655021,-19.6761655796569));
#52321=CARTESIAN_POINT('Ctrl Pts',(19.6605932821672,-16.5640988419222,-19.68034114387));
#52322=CARTESIAN_POINT('Ctrl Pts',(19.7378171886915,-16.597015700331,-19.684516708083));
#52323=CARTESIAN_POINT('Ctrl Pts',(19.81894148943,-16.6315951102716,-19.6889031700249));
#52324=CARTESIAN_POINT('Ctrl Pts',(19.8981843303164,-16.6703316765417,-19.6932896319667));
#52325=CARTESIAN_POINT('Ctrl Pts',(19.9751086547792,-16.7129713474294,-19.6976760939086));
#52326=CARTESIAN_POINT('Ctrl Pts',(20.0520329792421,-16.7556110183172,-19.7020625558505));
#52327=CARTESIAN_POINT('Ctrl Pts',(20.1266383352645,-16.8021534221799,-19.7064490177923));
#52328=CARTESIAN_POINT('Ctrl Pts',(20.1985254700754,-16.8522940330845,-19.7108354797342));
#52329=CARTESIAN_POINT('Ctrl Pts',(20.230696316323,-16.8747329004621,-19.7127985040371));
#52330=CARTESIAN_POINT('Ctrl Pts',(20.2623793611531,-16.8979308421821,-19.7147615283401));
#52331=CARTESIAN_POINT('Ctrl Pts',(20.293535888361,-16.9218650751948,-19.716724552643));
#52332=CARTESIAN_POINT('',(16.1740010149448,-18.9542795868247,-19.3667098901939));
#52333=CARTESIAN_POINT('Ctrl Pts',(16.1740010149441,-18.9542795861284,-19.3667098902285));
#52334=CARTESIAN_POINT('Ctrl Pts',(16.173926819566,-18.8709574030249,-19.3708480242598));
#52335=CARTESIAN_POINT('Ctrl Pts',(16.1779248169782,-18.7875513930795,-19.374986158291));
#52336=CARTESIAN_POINT('Ctrl Pts',(16.1859928190662,-18.7044936245066,-19.3791242923222));
#52337=CARTESIAN_POINT('Ctrl Pts',(16.1940571655296,-18.6214734895413,-19.3832605513584));
#52338=CARTESIAN_POINT('Ctrl Pts',(16.2061878113244,-18.5388017480886,-19.3873968103945));
#52339=CARTESIAN_POINT('Ctrl Pts',(16.2223305526747,-18.456907496146,-19.3915330694306));
#52340=CARTESIAN_POINT('Ctrl Pts',(16.238471016352,-18.3750247991377,-19.3956687448579));
#52341=CARTESIAN_POINT('Ctrl Pts',(16.2586223602409,-18.2939198329686,-19.3998044202853));
#52342=CARTESIAN_POINT('Ctrl Pts',(16.2826791433887,-18.2140121559657,-19.4039400957127));
#52343=CARTESIAN_POINT('Ctrl Pts',(16.3067400382202,-18.1340908214803,-19.4080764779922));
#52344=CARTESIAN_POINT('Ctrl Pts',(16.3347075604887,-18.0553676300741,-19.4122128602717));
#52345=CARTESIAN_POINT('Ctrl Pts',(16.3664266589084,-17.9782461940757,-19.4163492425513));
#52346=CARTESIAN_POINT('Ctrl Pts',(16.3981808282496,-17.9010394870584,-19.4204901983132));
#52347=CARTESIAN_POINT('Ctrl Pts',(16.4336946710468,-17.8254385023485,-19.4246311540751));
#52348=CARTESIAN_POINT('Ctrl Pts',(16.4727655806441,-17.7518254707252,-19.4287721098371));
#52349=CARTESIAN_POINT('Ctrl Pts',(16.511861777281,-17.6781647960941,-19.4329157456624));
#52350=CARTESIAN_POINT('Ctrl Pts',(16.5545193804023,-17.6064950352306,-19.4370593814876));
#52351=CARTESIAN_POINT('Ctrl Pts',(16.6004918491533,-17.5371703387789,-19.4412030173129));
#52352=CARTESIAN_POINT('Ctrl Pts',(16.6465392454185,-17.4677326545476,-19.4453534065787));
#52353=CARTESIAN_POINT('Ctrl Pts',(16.6959120078393,-17.4006480348314,-19.4495037958445));
#52354=CARTESIAN_POINT('Ctrl Pts',(16.7483230702929,-17.3362379102018,-19.4536541851102));
#52355=CARTESIAN_POINT('Ctrl Pts',(16.7661884610673,-17.3142823917967,-19.4550689308266));
#52356=CARTESIAN_POINT('Ctrl Pts',(16.7844065661398,-17.292637312599,-19.4564836765431));
#52357=CARTESIAN_POINT('Ctrl Pts',(16.8029650799467,-17.2713143846827,-19.4578984222595));
#52358=CARTESIAN_POINT('Ctrl Pts',(16.857858757406,-17.2082439287342,-19.4620830566462));
#52359=CARTESIAN_POINT('Ctrl Pts',(16.9159478005841,-17.1477482923964,-19.466267691033));
#52360=CARTESIAN_POINT('Ctrl Pts',(16.9769612646036,-17.0901689436695,-19.4704523254198));
#52361=CARTESIAN_POINT('Ctrl Pts',(17.0378878835037,-17.0326715520237,-19.4746310034971));
#52362=CARTESIAN_POINT('Ctrl Pts',(17.1017303233984,-16.9780825158866,-19.4788096815744));
#52363=CARTESIAN_POINT('Ctrl Pts',(17.1681782563647,-16.9267093376113,-19.4829883596517));
#52364=CARTESIAN_POINT('Ctrl Pts',(17.2358172209073,-16.8744153319337,-19.4872419375387));
#52365=CARTESIAN_POINT('Ctrl Pts',(17.306155687672,-16.8254539702902,-19.4914955154258));
#52366=CARTESIAN_POINT('Ctrl Pts',(17.3788280009098,-16.780109382846,-19.4957490933128));
#52367=CARTESIAN_POINT('Ctrl Pts',(17.4500914193922,-16.7356438888086,-19.4999202072833));
#52368=CARTESIAN_POINT('Ctrl Pts',(17.5235985912761,-16.6946564386902,-19.5040913212538));
#52369=CARTESIAN_POINT('Ctrl Pts',(17.5989738385239,-16.657372445741,-19.5082624352243));
#52370=CARTESIAN_POINT('Ctrl Pts',(17.6743237928742,-16.6201009637983,-19.5124321495369));
#52371=CARTESIAN_POINT('Ctrl Pts',(17.7515401656506,-16.5865306747361,-19.5166018638495));
#52372=CARTESIAN_POINT('Ctrl Pts',(17.8302229081151,-16.556840930505,-19.5207715781621));
#52373=CARTESIAN_POINT('Ctrl Pts',(17.9089028507045,-16.5271522427645,-19.5249411440981));
#52374=CARTESIAN_POINT('Ctrl Pts',(17.9890486285235,-16.5013439869149,-19.5291107100341));
#52375=CARTESIAN_POINT('Ctrl Pts',(18.0702417419427,-16.4795467699346,-19.53328027597));
#52376=CARTESIAN_POINT('Ctrl Pts',(18.1542895053979,-16.4569831896063,-19.5375964387176));
#52377=CARTESIAN_POINT('Ctrl Pts',(18.2394591140171,-16.4387180891091,-19.5419126014652));
#52378=CARTESIAN_POINT('Ctrl Pts',(18.3252730114503,-16.4248390932054,-19.5462287642128));
#52379=CARTESIAN_POINT('Ctrl Pts',(18.408291529862,-16.4114122041881,-19.5504043283958));
#52380=CARTESIAN_POINT('Ctrl Pts',(18.4919125329016,-16.402090058559,-19.5545798925788));
#52381=CARTESIAN_POINT('Ctrl Pts',(18.5756985998716,-16.3968990887408,-19.5587554567618));
#52382=CARTESIAN_POINT('Ctrl Pts',(18.6637165024314,-16.3914459353448,-19.5631419187917));
#52383=CARTESIAN_POINT('Ctrl Pts',(18.75191599805,-16.3905522627807,-19.5675283808215));
#52384=CARTESIAN_POINT('Ctrl Pts',(18.8397925195445,-16.3941868827437,-19.5719148428514));
#52385=CARTESIAN_POINT('Ctrl Pts',(18.927669041039,-16.3978215027067,-19.5763013048812));
#52386=CARTESIAN_POINT('Ctrl Pts',(19.0152220177589,-16.4059842855989,-19.580687766911));
#52387=CARTESIAN_POINT('Ctrl Pts',(19.1019580505821,-16.4185819782334,-19.5850742289409));
#52388=CARTESIAN_POINT('Ctrl Pts',(19.1847019893314,-16.4305998521642,-19.5892588006086));
#52389=CARTESIAN_POINT('Ctrl Pts',(19.267010516095,-16.4466981015606,-19.5934433722764));
#52390=CARTESIAN_POINT('Ctrl Pts',(19.3484498725052,-16.4668337371157,-19.5976279439441));
#52391=CARTESIAN_POINT('Ctrl Pts',(19.433563152438,-16.4878777391949,-19.602001291616));
#52392=CARTESIAN_POINT('Ctrl Pts',(19.5177264872397,-16.5133320197713,-19.6063746392878));
#52393=CARTESIAN_POINT('Ctrl Pts',(19.6004511653704,-16.5430868886512,-19.6107479869597));
#52394=CARTESIAN_POINT('Ctrl Pts',(19.6793978237086,-16.571482858517,-19.6149216047029));
#52395=CARTESIAN_POINT('Ctrl Pts',(19.7570338500724,-16.6037950595409,-19.619095222446));
#52396=CARTESIAN_POINT('Ctrl Pts',(19.8329471640918,-16.6398764889101,-19.6232688401892));
#52397=CARTESIAN_POINT('Ctrl Pts',(19.9088089339765,-16.6759334194668,-19.6274396241012));
#52398=CARTESIAN_POINT('Ctrl Pts',(19.9829499008247,-16.7157542975669,-19.6316104080133));
#52399=CARTESIAN_POINT('Ctrl Pts',(20.0549778822146,-16.7591440004643,-19.6357811919253));
#52400=CARTESIAN_POINT('Ctrl Pts',(20.1269801310666,-16.8025182020641,-19.6399504857934));
#52401=CARTESIAN_POINT('Ctrl Pts',(20.1968705010822,-16.849458457535,-19.6441197796615));
#52402=CARTESIAN_POINT('Ctrl Pts',(20.2642825299598,-16.8997243414931,-19.6482890735296));
#52403=CARTESIAN_POINT('Ctrl Pts',(20.2740863758758,-16.9070345944162,-19.6488954210219));
#52404=CARTESIAN_POINT('Ctrl Pts',(20.2838378536473,-16.9144151106639,-19.6495017685142));
#52405=CARTESIAN_POINT('Ctrl Pts',(20.293535888361,-16.9218650751947,-19.6501081160065));
#52406=CARTESIAN_POINT('Ctrl Pts',(20.293535888361,-16.9218650751948,-18.8501886412182));
#52407=CARTESIAN_POINT('Ctrl Pts',(20.3600880992579,-16.9729900324945,-18.8543616964033));
#52408=CARTESIAN_POINT('Ctrl Pts',(20.4241919589121,-17.0274434638868,-18.8585347515884));
#52409=CARTESIAN_POINT('Ctrl Pts',(20.4855007810524,-17.0849582184716,-18.8627078067735));
#52410=CARTESIAN_POINT('Ctrl Pts',(20.5467748089402,-17.1424403320298,-18.866878493648));
#52411=CARTESIAN_POINT('Ctrl Pts',(20.6052566139188,-17.2029800053482,-18.8710491805225));
#52412=CARTESIAN_POINT('Ctrl Pts',(20.6606332981064,-17.2662704443987,-18.8752198673969));
#52413=CARTESIAN_POINT('Ctrl Pts',(20.7159951665402,-17.3295439504101,-18.8793894384251));
#52414=CARTESIAN_POINT('Ctrl Pts',(20.7682532615728,-17.3955664142886,-18.8835590094532));
#52415=CARTESIAN_POINT('Ctrl Pts',(20.8171331656151,-17.4639958957334,-18.8877285804813));
#52416=CARTESIAN_POINT('Ctrl Pts',(20.8660146547938,-17.5324275962917,-18.8918982867253));
#52417=CARTESIAN_POINT('Ctrl Pts',(20.9115174691059,-17.6032660943068,-18.8960679929693));
#52418=CARTESIAN_POINT('Ctrl Pts',(20.9534097498297,-17.6761393640524,-18.9002376992133));
#52419=CARTESIAN_POINT('Ctrl Pts',(20.995344766866,-17.7490869752939,-18.9044116591734));
#52420=CARTESIAN_POINT('Ctrl Pts',(21.033661663671,-17.8240731045976,-18.9085856191335));
#52421=CARTESIAN_POINT('Ctrl Pts',(21.068174170418,-17.9007003556771,-18.9127595790936));
#52422=CARTESIAN_POINT('Ctrl Pts',(21.1027039969298,-17.9773660613949,-18.9169356337148));
#52423=CARTESIAN_POINT('Ctrl Pts',(21.1334254624243,-18.055674100626,-18.9211116883359));
#52424=CARTESIAN_POINT('Ctrl Pts',(21.1602010986746,-18.1352085769364,-18.9252877429571));
#52425=CARTESIAN_POINT('Ctrl Pts',(21.1870245435949,-18.2148850643459,-18.9294712540441));
#52426=CARTESIAN_POINT('Ctrl Pts',(21.2098879571468,-18.295791920553,-18.9336547651311));
#52427=CARTESIAN_POINT('Ctrl Pts',(21.2287042787308,-18.377499728736,-18.9378382762182));
#52428=CARTESIAN_POINT('Ctrl Pts',(21.2457310808275,-18.4514367452501,-18.94162391599));
#52429=CARTESIAN_POINT('Ctrl Pts',(21.2594446082458,-18.5260292265647,-18.9454095557619));
#52430=CARTESIAN_POINT('Ctrl Pts',(21.2698170137415,-18.6009557395155,-18.9491951955337));
#52431=CARTESIAN_POINT('Ctrl Pts',(21.2812826384042,-18.6837792730856,-18.9533798299225));
#52432=CARTESIAN_POINT('Ctrl Pts',(21.2887076244828,-18.7673192548721,-18.9575644643113));
#52433=CARTESIAN_POINT('Ctrl Pts',(21.2920126435715,-18.851147060883,-18.9617490987001));
#52434=CARTESIAN_POINT('Ctrl Pts',(21.2953129583745,-18.934855548388,-18.9659277767799));
#52435=CARTESIAN_POINT('Ctrl Pts',(21.294504936491,-19.0188505906155,-18.9701064548596));
#52436=CARTESIAN_POINT('Ctrl Pts',(21.2895607321101,-19.1026961993451,-18.9742851329393));
#52437=CARTESIAN_POINT('Ctrl Pts',(21.2845279064127,-19.1880446804597,-18.9785387108258));
#52438=CARTESIAN_POINT('Ctrl Pts',(21.2752090914542,-19.2732378406073,-18.9827922887123));
#52439=CARTESIAN_POINT('Ctrl Pts',(21.2616304174303,-19.3578133473421,-18.9870458665988));
#52440=CARTESIAN_POINT('Ctrl Pts',(21.2483149925156,-19.4407491927399,-18.9912169805726));
#52441=CARTESIAN_POINT('Ctrl Pts',(21.2309034822292,-19.5230906447102,-18.9953880945464));
#52442=CARTESIAN_POINT('Ctrl Pts',(21.2094728610011,-19.6044064028251,-18.9995592085202));
#52443=CARTESIAN_POINT('Ctrl Pts',(21.1880494310247,-19.6856948746526,-19.0037289228364));
#52444=CARTESIAN_POINT('Ctrl Pts',(21.1626096856898,-19.7659578917013,-19.0078986371526));
#52445=CARTESIAN_POINT('Ctrl Pts',(21.1332813336496,-19.8447760536666,-19.0120683514689));
#52446=CARTESIAN_POINT('Ctrl Pts',(21.1039540252378,-19.9235914109442,-19.0162379174088));
#52447=CARTESIAN_POINT('Ctrl Pts',(21.0707385464732,-20.0009615845084,-19.0204074833488));
#52448=CARTESIAN_POINT('Ctrl Pts',(21.0338114728018,-20.0764852998459,-19.0245770492887));
#52449=CARTESIAN_POINT('Ctrl Pts',(20.9955860886931,-20.1546643360123,-19.0288932120326));
#52450=CARTESIAN_POINT('Ctrl Pts',(20.9533834858384,-20.2308641813314,-19.0332093747765));
#52451=CARTESIAN_POINT('Ctrl Pts',(20.9074514472649,-20.3046672933068,-19.0375255375203));
#52452=CARTESIAN_POINT('Ctrl Pts',(20.8630156401099,-20.3760662765228,-19.041701101708));
#52453=CARTESIAN_POINT('Ctrl Pts',(20.815089945817,-20.4452219153955,-19.0458766658958));
#52454=CARTESIAN_POINT('Ctrl Pts',(20.7639418957712,-20.5117871328463,-19.0500522300835));
#52455=CARTESIAN_POINT('Ctrl Pts',(20.7102104791443,-20.5817144014031,-19.0544386921054));
#52456=CARTESIAN_POINT('Ctrl Pts',(20.6529230087043,-20.6487822429891,-19.0588251541274));
#52457=CARTESIAN_POINT('Ctrl Pts',(20.5924345734849,-20.7126308346942,-19.0632116161493));
#52458=CARTESIAN_POINT('Ctrl Pts',(20.5319461382654,-20.7764794263994,-19.0675980781712));
#52459=CARTESIAN_POINT('Ctrl Pts',(20.4682572109593,-20.837108423261,-19.0719845401932));
#52460=CARTESIAN_POINT('Ctrl Pts',(20.4017623229462,-20.8942072068039,-19.0763710022151));
#52461=CARTESIAN_POINT('Ctrl Pts',(20.3383269634742,-20.9486787905254,-19.0805556366056));
#52462=CARTESIAN_POINT('Ctrl Pts',(20.2721020634022,-21.0001406364731,-19.0847402709961));
#52463=CARTESIAN_POINT('Ctrl Pts',(20.2034050887149,-21.0482940359737,-19.0889249053866));
#52464=CARTESIAN_POINT('Ctrl Pts',(20.1348058956689,-21.0963788950696,-19.093103583468));
#52465=CARTESIAN_POINT('Ctrl Pts',(20.0637419907205,-21.141164399806,-19.0972822615493));
#52466=CARTESIAN_POINT('Ctrl Pts',(19.990564898557,-21.1823911441078,-19.1014609396307));
#52467=CARTESIAN_POINT('Ctrl Pts',(19.9160761595504,-21.2243568482045,-19.1057145175168));
#52468=CARTESIAN_POINT('Ctrl Pts',(19.8393980962008,-21.2626346413139,-19.1099680954028));
#52469=CARTESIAN_POINT('Ctrl Pts',(19.7609336007081,-21.2969962430112,-19.1142216732889));
#52470=CARTESIAN_POINT('Ctrl Pts',(19.683990292633,-21.3306916779815,-19.1183927872642));
#52471=CARTESIAN_POINT('Ctrl Pts',(19.6053296420408,-21.360621219484,-19.1225639012394));
#52472=CARTESIAN_POINT('Ctrl Pts',(19.5253559691356,-21.3866161360907,-19.1267350152147));
#52473=CARTESIAN_POINT('Ctrl Pts',(19.4454091321695,-21.412602329852,-19.1309047295323));
#52474=CARTESIAN_POINT('Ctrl Pts',(19.3641505850609,-21.4346563787685,-19.1350744438499));
#52475=CARTESIAN_POINT('Ctrl Pts',(19.2820021033665,-21.4526586521766,-19.1392441581676));
#52476=CARTESIAN_POINT('Ctrl Pts',(19.1998565448683,-21.4706602849865,-19.1434137241088));
#52477=CARTESIAN_POINT('Ctrl Pts',(19.1168215642993,-21.4846103313103,-19.1475832900501));
#52478=CARTESIAN_POINT('Ctrl Pts',(19.0333301469624,-21.4944400608706,-19.1517528559914));
#52479=CARTESIAN_POINT('Ctrl Pts',(18.9469032742685,-21.5046153916102,-19.1560690187335));
#52480=CARTESIAN_POINT('Ctrl Pts',(18.8599877947896,-21.5103752123296,-19.1603851814756));
#52481=CARTESIAN_POINT('Ctrl Pts',(18.7730689159398,-21.511701861508,-19.1647013442177));
#52482=CARTESIAN_POINT('Ctrl Pts',(18.688981410545,-21.512985295227,-19.1688769084066));
#52483=CARTESIAN_POINT('Ctrl Pts',(18.6048911930078,-21.510120006403,-19.1730524725954));
#52484=CARTESIAN_POINT('Ctrl Pts',(18.5212349098899,-21.5031430803525,-19.1772280367843));
#52485=CARTESIAN_POINT('Ctrl Pts',(18.4333533466026,-21.495813766338,-19.181614498803));
#52486=CARTESIAN_POINT('Ctrl Pts',(18.3459512843982,-21.4839466202446,-19.1860009608217));
#52487=CARTESIAN_POINT('Ctrl Pts',(18.2595234803591,-21.467645450438,-19.1903874228405));
#52488=CARTESIAN_POINT('Ctrl Pts',(18.1730956763199,-21.4513442806314,-19.1947738848592));
#52489=CARTESIAN_POINT('Ctrl Pts',(18.0876426763647,-21.4306092978499,-19.1991603468779));
#52490=CARTESIAN_POINT('Ctrl Pts',(18.0036392138265,-21.4056041086573,-19.2035468088966));
#52491=CARTESIAN_POINT('Ctrl Pts',(17.9235008748327,-21.3817494451997,-19.2077314433107));
#52492=CARTESIAN_POINT('Ctrl Pts',(17.8443833236107,-21.3539201055369,-19.2119160777248));
#52493=CARTESIAN_POINT('Ctrl Pts',(17.7667095652025,-21.3222213429866,-19.2161007121389));
#52494=CARTESIAN_POINT('Ctrl Pts',(17.6891463657735,-21.2905676997005,-19.2202793902439));
#52495=CARTESIAN_POINT('Ctrl Pts',(17.6130232994484,-21.2550557457776,-19.224458068349));
#52496=CARTESIAN_POINT('Ctrl Pts',(17.5387487593335,-21.2158406462658,-19.228636746454));
#52497=CARTESIAN_POINT('Ctrl Pts',(17.4631429019428,-21.1759226445297,-19.2328903243342));
#52498=CARTESIAN_POINT('Ctrl Pts',(17.3894529543292,-21.1321675712374,-19.2371439022144));
#52499=CARTESIAN_POINT('Ctrl Pts',(17.3180889421044,-21.0847906311049,-19.2413974800945));
#52500=CARTESIAN_POINT('Ctrl Pts',(17.2481084600712,-21.0383321851128,-19.2455685940936));
#52501=CARTESIAN_POINT('Ctrl Pts',(17.1803649335769,-20.9883913190988,-19.2497397080926));
#52502=CARTESIAN_POINT('Ctrl Pts',(17.1152190899104,-20.9352166712514,-19.2539108220917));
#52503=CARTESIAN_POINT('Ctrl Pts',(17.0500951065615,-20.882059866671,-19.2580805364331));
#52504=CARTESIAN_POINT('Ctrl Pts',(16.987567430963,-20.8256717259896,-19.2622502507746));
#52505=CARTESIAN_POINT('Ctrl Pts',(16.9279649526829,-20.7663421418967,-19.266419965116));
#52506=CARTESIAN_POINT('Ctrl Pts',(16.8683645953157,-20.707014669006,-19.270589531081));
#52507=CARTESIAN_POINT('Ctrl Pts',(16.8116895537436,-20.6447462859623,-19.2747590970461));
#52508=CARTESIAN_POINT('Ctrl Pts',(16.7582319859876,-20.5798638624914,-19.2789286630111));
#52509=CARTESIAN_POINT('Ctrl Pts',(16.7028949166956,-20.5127002537798,-19.283244825725));
#52510=CARTESIAN_POINT('Ctrl Pts',(16.6510061189315,-20.4427357723036,-19.2875609884389));
#52511=CARTESIAN_POINT('Ctrl Pts',(16.6028430768027,-20.370368840855,-19.2918771511528));
#52512=CARTESIAN_POINT('Ctrl Pts',(16.5562489402056,-20.3003592538356,-19.2960527153651));
#52513=CARTESIAN_POINT('Ctrl Pts',(16.5131417547233,-20.2281017614849,-19.3002282795774));
#52514=CARTESIAN_POINT('Ctrl Pts',(16.4737266859787,-20.1539835880423,-19.3044038437897));
#52515=CARTESIAN_POINT('Ctrl Pts',(16.4323208564678,-20.0761218830912,-19.3087903057544));
#52516=CARTESIAN_POINT('Ctrl Pts',(16.3949901703475,-19.9962071202823,-19.3131767677191));
#52517=CARTESIAN_POINT('Ctrl Pts',(16.3619151438293,-19.9147115015028,-19.3175632296838));
#52518=CARTESIAN_POINT('Ctrl Pts',(16.3288401173112,-19.8332158827234,-19.3219496916486));
#52519=CARTESIAN_POINT('Ctrl Pts',(16.3000208686933,-19.7501399810729,-19.3263361536133));
#52520=CARTESIAN_POINT('Ctrl Pts',(16.2755767948947,-19.6659715292643,-19.330722615578));
#52521=CARTESIAN_POINT('Ctrl Pts',(16.2465257453528,-19.5659398453678,-19.3359357942364));
#52522=CARTESIAN_POINT('Ctrl Pts',(16.2235642356486,-19.464065347825,-19.3411489728948));
#52523=CARTESIAN_POINT('Ctrl Pts',(16.2068848499427,-19.3610098022674,-19.3463621515532));
#52524=CARTESIAN_POINT('Ctrl Pts',(16.1904712789856,-19.2595966243872,-19.3514922492277));
#52525=CARTESIAN_POINT('Ctrl Pts',(16.1801412137013,-19.1570396545395,-19.3566223469021));
#52526=CARTESIAN_POINT('Ctrl Pts',(16.1760324691903,-19.0539907413612,-19.3617524445766));
#52527=CARTESIAN_POINT('Ctrl Pts',(16.1747089805837,-19.0207971314519,-19.363404926449));
#52528=CARTESIAN_POINT('Ctrl Pts',(16.1740306434087,-18.9875526505075,-19.3650574083215));
#52529=CARTESIAN_POINT('Ctrl Pts',(16.1740010149447,-18.9542795868247,-19.3667098901939));
#52530=CARTESIAN_POINT('Origin',(18.734,-18.952,1.76670989022851));
#52531=CARTESIAN_POINT('',(20.293535888361,-16.9218650751948,-18.0500683203253));
#52532=CARTESIAN_POINT('',(20.293535888361,-16.9218650751948,-18.1167065567592));
#52533=CARTESIAN_POINT('',(20.293535888361,-16.9218650751948,1.76670989022851));
#52534=CARTESIAN_POINT('',(16.1743944468539,-18.9516176052701,-18.6332901348849));
#52535=CARTESIAN_POINT('Ctrl Pts',(20.293535888361,-16.9218650751948,-18.1167065567592));
#52536=CARTESIAN_POINT('Ctrl Pts',(20.3602206256079,-16.9730918383383,-18.1208760361824));
#52537=CARTESIAN_POINT('Ctrl Pts',(20.4243870824807,-17.0276141077345,-18.1250455156056));
#52538=CARTESIAN_POINT('Ctrl Pts',(20.4857019893154,-17.0851469954417,-18.1292149950289));
#52539=CARTESIAN_POINT('Ctrl Pts',(20.5470276420194,-17.1426899661927,-18.1333852051827));
#52540=CARTESIAN_POINT('Ctrl Pts',(20.6055004178084,-17.2032442872454,-18.1375554153366));
#52541=CARTESIAN_POINT('Ctrl Pts',(20.6608233620813,-17.2664876946941,-18.1417256254905));
#52542=CARTESIAN_POINT('Ctrl Pts',(20.7162074135451,-17.3298009579145,-18.1459004418675));
#52543=CARTESIAN_POINT('Ctrl Pts',(20.7684343867049,-17.3958088885422,-18.1500752582446));
#52544=CARTESIAN_POINT('Ctrl Pts',(20.8172475188104,-17.464155997636,-18.1542500746216));
#52545=CARTESIAN_POINT('Ctrl Pts',(20.8660913992488,-17.5325461598914,-18.158427520796));
#52546=CARTESIAN_POINT('Ctrl Pts',(20.9115169101421,-17.60327804657,-18.1626049669703));
#52547=CARTESIAN_POINT('Ctrl Pts',(20.953311845506,-17.6759690707523,-18.1667824131447));
#52548=CARTESIAN_POINT('Ctrl Pts',(20.995175289534,-17.7487792472892,-18.1709667068295));
#52549=CARTESIAN_POINT('Ctrl Pts',(21.0333960713853,-17.82355456178,-18.1751510005143));
#52550=CARTESIAN_POINT('Ctrl Pts',(21.0678091437387,-17.8998902715962,-18.1793352941991));
#52551=CARTESIAN_POINT('Ctrl Pts',(21.0825869345977,-17.9326706389858,-18.1811321293184));
#52552=CARTESIAN_POINT('Ctrl Pts',(21.0966631843942,-17.9657385349447,-18.1829289644377));
#52553=CARTESIAN_POINT('Ctrl Pts',(21.1100276507034,-17.9990610706384,-18.184725799557));
#52554=CARTESIAN_POINT('Ctrl Pts',(21.1411520453503,-18.0766656473997,-18.1889104339505));
#52555=CARTESIAN_POINT('Ctrl Pts',(21.1685283427045,-18.1559410996702,-18.193095068344));
#52556=CARTESIAN_POINT('Ctrl Pts',(21.1919760688458,-18.2364906394873,-18.1972797027375));
#52557=CARTESIAN_POINT('Ctrl Pts',(21.2153904200512,-18.3169255270045,-18.2014583808218));
#52558=CARTESIAN_POINT('Ctrl Pts',(21.2348871797097,-18.3986304619535,-18.2056370589062));
#52559=CARTESIAN_POINT('Ctrl Pts',(21.2503340551361,-18.4811890793937,-18.2098157369906));
#52560=CARTESIAN_POINT('Ctrl Pts',(21.2660578047011,-18.5652275007066,-18.2140693148759));
#52561=CARTESIAN_POINT('Ctrl Pts',(21.2775848741471,-18.6501500625618,-18.2183228927613));
#52562=CARTESIAN_POINT('Ctrl Pts',(21.2848289888802,-18.7355018025751,-18.2225764706466));
#52563=CARTESIAN_POINT('Ctrl Pts',(21.2919326623144,-18.819198832569,-18.226747584625));
#52564=CARTESIAN_POINT('Ctrl Pts',(21.2949179252555,-18.9033080688148,-18.2309186986034));
#52565=CARTESIAN_POINT('Ctrl Pts',(21.2937553357682,-18.9873923862785,-18.2350898125818));
#52566=CARTESIAN_POINT('Ctrl Pts',(21.2925931363989,-19.0714484884373,-18.2392595269026));
#52567=CARTESIAN_POINT('Ctrl Pts',(21.287285855196,-19.1554792288145,-18.2434292412234));
#52568=CARTESIAN_POINT('Ctrl Pts',(21.2778561566697,-19.2390467804623,-18.2475989555442));
#52569=CARTESIAN_POINT('Ctrl Pts',(21.2684267936925,-19.3226113584179,-18.2517685214887));
#52570=CARTESIAN_POINT('Ctrl Pts',(21.2548753574853,-19.4057123233788,-18.2559380874332));
#52571=CARTESIAN_POINT('Ctrl Pts',(21.2372763100333,-19.4879176388457,-18.2601076533776));
#52572=CARTESIAN_POINT('Ctrl Pts',(21.2190585017878,-19.5730131917741,-18.264423816116));
#52573=CARTESIAN_POINT('Ctrl Pts',(21.1965032689152,-19.6571484255578,-18.2687399788544));
#52574=CARTESIAN_POINT('Ctrl Pts',(21.1697502461668,-19.7398583237475,-18.2730561415928));
#52575=CARTESIAN_POINT('Ctrl Pts',(21.1438687003148,-19.819873955721,-18.2772317057849));
#52576=CARTESIAN_POINT('Ctrl Pts',(21.1140588617648,-19.8985552629124,-18.281407269977));
#52577=CARTESIAN_POINT('Ctrl Pts',(21.0804965434243,-19.9755008410831,-18.2855828341691));
#52578=CARTESIAN_POINT('Ctrl Pts',(21.0452390721828,-20.0563327574599,-18.2899692961807));
#52579=CARTESIAN_POINT('Ctrl Pts',(21.0058403441651,-20.1352484709672,-18.2943557581922));
#52580=CARTESIAN_POINT('Ctrl Pts',(20.9625580617869,-20.2118130675798,-18.2987422202038));
#52581=CARTESIAN_POINT('Ctrl Pts',(20.9192757794087,-20.2883776641924,-18.3031286822153));
#52582=CARTESIAN_POINT('Ctrl Pts',(20.8721103180846,-20.3625906950211,-18.3075151442269));
#52583=CARTESIAN_POINT('Ctrl Pts',(20.8213695361433,-20.4340554711552,-18.3119016062384));
#52584=CARTESIAN_POINT('Ctrl Pts',(20.7729634127897,-20.5022320470106,-18.3160862406309));
#52585=CARTESIAN_POINT('Ctrl Pts',(20.7211235735796,-20.5681614794158,-18.3202708750235));
#52586=CARTESIAN_POINT('Ctrl Pts',(20.6660859672863,-20.6314772445661,-18.324455509416));
#52587=CARTESIAN_POINT('Ctrl Pts',(20.6111267002133,-20.6947028875616,-18.3286341874995));
#52588=CARTESIAN_POINT('Ctrl Pts',(20.5529790062393,-20.7553219086264,-18.3328128655829));
#52589=CARTESIAN_POINT('Ctrl Pts',(20.4919213748666,-20.8129977001026,-18.3369915436664));
#52590=CARTESIAN_POINT('Ctrl Pts',(20.4297693293237,-20.8717072886989,-18.3412451215519));
#52591=CARTESIAN_POINT('Ctrl Pts',(20.3646022781503,-20.9273667019604,-18.3454986994375));
#52592=CARTESIAN_POINT('Ctrl Pts',(20.2967560739107,-20.9796571340972,-18.3497522773231));
#52593=CARTESIAN_POINT('Ctrl Pts',(20.2302252007411,-21.0309338141631,-18.3539233913005));
#52594=CARTESIAN_POINT('Ctrl Pts',(20.1611185098595,-21.0789706821842,-18.358094505278));
#52595=CARTESIAN_POINT('Ctrl Pts',(20.0897876178816,-21.1235063746623,-18.3622656192554));
#52596=CARTESIAN_POINT('Ctrl Pts',(20.0184806616733,-21.1680271227587,-18.3664353335753));
#52597=CARTESIAN_POINT('Ctrl Pts',(19.9449513765315,-21.2090487851565,-18.3706050478952));
#52598=CARTESIAN_POINT('Ctrl Pts',(19.8695801735013,-21.2463534316994,-18.3747747622151));
#52599=CARTESIAN_POINT('Ctrl Pts',(19.7942116525019,-21.2836567507829,-18.3789443281586));
#52600=CARTESIAN_POINT('Ctrl Pts',(19.7170017566051,-21.3172431136927,-18.3831138941022));
#52601=CARTESIAN_POINT('Ctrl Pts',(19.6383540649958,-21.346941278012,-18.3872834600458));
#52602=CARTESIAN_POINT('Ctrl Pts',(19.5569412175515,-21.3776835931598,-18.3915996227853));
#52603=CARTESIAN_POINT('Ctrl Pts',(19.473988080848,-21.4042590180671,-18.3959157855248));
#52604=CARTESIAN_POINT('Ctrl Pts',(19.3899612417722,-21.4265332588779,-18.4002319482643));
#52605=CARTESIAN_POINT('Ctrl Pts',(19.3086715681612,-21.4480819186317,-18.4044075124555));
#52606=CARTESIAN_POINT('Ctrl Pts',(19.2263775401996,-21.4656052611968,-18.4085830766467));
#52607=CARTESIAN_POINT('Ctrl Pts',(19.1435118395205,-21.4790338449045,-18.4127586408379));
#52608=CARTESIAN_POINT('Ctrl Pts',(19.0564607892627,-21.4931406744569,-18.4171451028516));
#52609=CARTESIAN_POINT('Ctrl Pts',(18.9687793786242,-21.5027281581545,-18.4215315648652));
#52610=CARTESIAN_POINT('Ctrl Pts',(18.8809727909042,-21.5077775722339,-18.4259180268789));
#52611=CARTESIAN_POINT('Ctrl Pts',(18.7931662031843,-21.5128269863133,-18.4303044888925));
#52612=CARTESIAN_POINT('Ctrl Pts',(18.7052350190324,-21.5133384034635,-18.4346909509062));
#52613=CARTESIAN_POINT('Ctrl Pts',(18.6176794289205,-21.5093559636358,-18.4390774129198));
#52614=CARTESIAN_POINT('Ctrl Pts',(18.5341524013308,-21.5055567617695,-18.4432620473123));
#52615=CARTESIAN_POINT('Ctrl Pts',(18.4506562604967,-21.4976540121365,-18.4474466817048));
#52616=CARTESIAN_POINT('Ctrl Pts',(18.3676269095303,-21.4856477179315,-18.4516313160972));
#52617=CARTESIAN_POINT('Ctrl Pts',(18.2847157405683,-21.4736585132003,-18.4558099941806));
#52618=CARTESIAN_POINT('Ctrl Pts',(18.2022704931348,-21.4575774310126,-18.4599886722639));
#52619=CARTESIAN_POINT('Ctrl Pts',(18.1207249420861,-21.4374564376268,-18.4641673503473));
#52620=CARTESIAN_POINT('Ctrl Pts',(18.0377177456259,-21.4169747898918,-18.4684209282329));
#52621=CARTESIAN_POINT('Ctrl Pts',(17.9556432985576,-21.3923069974989,-18.4726745061184));
#52622=CARTESIAN_POINT('Ctrl Pts',(17.8749514567215,-21.3635628957776,-18.476928084004));
#52623=CARTESIAN_POINT('Ctrl Pts',(17.7958239837108,-21.3353760545626,-18.4810991979814));
#52624=CARTESIAN_POINT('Ctrl Pts',(17.7180264386448,-21.3032697094722,-18.4852703119587));
#52625=CARTESIAN_POINT('Ctrl Pts',(17.6419689102691,-21.267398043331,-18.4894414259361));
#52626=CARTESIAN_POINT('Ctrl Pts',(17.5659369037317,-21.2315384142739,-18.4936111402558));
#52627=CARTESIAN_POINT('Ctrl Pts',(17.4916441700223,-21.1919161695519,-18.4977808545756));
#52628=CARTESIAN_POINT('Ctrl Pts',(17.4194798631977,-21.1487332131921,-18.5019505688954));
#52629=CARTESIAN_POINT('Ctrl Pts',(17.347318124289,-21.1055517934674,-18.5061201348388));
#52630=CARTESIAN_POINT('Ctrl Pts',(17.2772850559936,-21.0588101509788,-18.5102897007822));
#52631=CARTESIAN_POINT('Ctrl Pts',(17.2097430958425,-21.0087549416807,-18.5144592667256));
#52632=CARTESIAN_POINT('Ctrl Pts',(17.1398264436723,-20.9569398529571,-18.5187754294653));
#52633=CARTESIAN_POINT('Ctrl Pts',(17.0725797574076,-20.9015741660664,-18.5230915922049));
#52634=CARTESIAN_POINT('Ctrl Pts',(17.0083685115613,-20.8429775160242,-18.5274077549445));
#52635=CARTESIAN_POINT('Ctrl Pts',(16.9462489403141,-20.7862896457115,-18.5315833191356));
#52636=CARTESIAN_POINT('Ctrl Pts',(16.886970385841,-20.7265784444844,-18.5357588833267));
#52637=CARTESIAN_POINT('Ctrl Pts',(16.8308254399578,-20.6641701416647,-18.5399344475178));
#52638=CARTESIAN_POINT('Ctrl Pts',(16.7718447463027,-20.598609743801,-18.5443209095317));
#52639=CARTESIAN_POINT('Ctrl Pts',(16.7163229051915,-20.5300730764182,-18.5487073715456));
#52640=CARTESIAN_POINT('Ctrl Pts',(16.6645491064847,-20.4589747839061,-18.5530938335595));
#52641=CARTESIAN_POINT('Ctrl Pts',(16.6127753077778,-20.3878764913939,-18.5574802955735));
#52642=CARTESIAN_POINT('Ctrl Pts',(16.5647498046499,-20.3142171013321,-18.5618667575874));
#52643=CARTESIAN_POINT('Ctrl Pts',(16.5207062260026,-20.2384410868689,-18.5662532196013));
#52644=CARTESIAN_POINT('Ctrl Pts',(16.4770273612297,-20.1632925546556,-18.5706033584189));
#52645=CARTESIAN_POINT('Ctrl Pts',(16.4371122169919,-20.0858014915384,-18.5749534972364));
#52646=CARTESIAN_POINT('Ctrl Pts',(16.4012086273382,-20.0063644586359,-18.579303636054));
#52647=CARTESIAN_POINT('Ctrl Pts',(16.3640774712897,-19.924211423433,-18.5838025088638));
#52648=CARTESIAN_POINT('Ctrl Pts',(16.3312374248383,-19.8399772763342,-18.5883013816736));
#52649=CARTESIAN_POINT('Ctrl Pts',(16.3029130373491,-19.7541322709061,-18.5928002544834));
#52650=CARTESIAN_POINT('Ctrl Pts',(16.2756354411693,-19.6714598603193,-18.5971328613515));
#52651=CARTESIAN_POINT('Ctrl Pts',(16.252545805577,-19.5872939815205,-18.6014654682196));
#52652=CARTESIAN_POINT('Ctrl Pts',(16.2337970621825,-19.5020775124732,-18.6057980750876));
#52653=CARTESIAN_POINT('Ctrl Pts',(16.2150725182341,-19.416971034336,-18.6101250897577));
#52654=CARTESIAN_POINT('Ctrl Pts',(16.2006778102741,-19.3308170607077,-18.6144521044277));
#52655=CARTESIAN_POINT('Ctrl Pts',(16.190716084581,-19.244073493441,-18.6187791190978));
#52656=CARTESIAN_POINT('Ctrl Pts',(16.180768168227,-19.1574501735471,-18.6231001354885));
#52657=CARTESIAN_POINT('Ctrl Pts',(16.1752410444518,-19.0702392928349,-18.6274211518792));
#52658=CARTESIAN_POINT('Ctrl Pts',(16.1741865858058,-18.9829076772249,-18.6317421682699));
#52659=CARTESIAN_POINT('Ctrl Pts',(16.1740606709629,-18.9724792486655,-18.6322581487704));
#52660=CARTESIAN_POINT('Ctrl Pts',(16.1739984722012,-18.9620491070313,-18.632774129271));
#52661=CARTESIAN_POINT('Ctrl Pts',(16.1740000284928,-18.9516180532909,-18.6332901097715));
#52662=CARTESIAN_POINT('Ctrl Pts',(16.178162963747,-18.9516133246024,-18.6332903748342));
#52663=CARTESIAN_POINT('Ctrl Pts',(16.1776269370726,-18.5470182282415,-18.6533365919837));
#52664=CARTESIAN_POINT('Ctrl Pts',(16.4590847030962,-17.2875284349863,-18.7157747446936));
#52665=CARTESIAN_POINT('Ctrl Pts',(18.2370603661219,-16.0736326739786,-18.8102032534018));
#52666=CARTESIAN_POINT('Ctrl Pts',(19.7793305886778,-16.5353973209162,-18.8845855449605));
#52667=CARTESIAN_POINT('Ctrl Pts',(20.2933494025375,-16.9221164381226,-18.9165759009586));
#52668=CARTESIAN_POINT('',(16.1740000028035,-18.9518801919504,-18.5667098901964));
#52669=CARTESIAN_POINT('Ctrl Pts',(16.1740000028035,-18.9518801913083,-18.5667098902285));
#52670=CARTESIAN_POINT('Ctrl Pts',(16.1740003013853,-18.945500276023,-18.5670291853155));
#52671=CARTESIAN_POINT('Ctrl Pts',(16.1740244495167,-18.9391204260769,-18.5673484804024));
#52672=CARTESIAN_POINT('Ctrl Pts',(16.1740724460423,-18.9327407557765,-18.5676677754894));
#52673=CARTESIAN_POINT('Ctrl Pts',(16.1747014814392,-18.8491297362399,-18.5718524098819));
#52674=CARTESIAN_POINT('Ctrl Pts',(16.1794322843349,-18.7653939703416,-18.5760370442745));
#52675=CARTESIAN_POINT('Ctrl Pts',(16.1882813814472,-18.6819690477863,-18.580221678667));
#52676=CARTESIAN_POINT('Ctrl Pts',(16.1971178829649,-18.5986628702823,-18.5844003567505));
#52677=CARTESIAN_POINT('Ctrl Pts',(16.2100609870472,-18.515667110836,-18.5885790348339));
#52678=CARTESIAN_POINT('Ctrl Pts',(16.2270752140172,-18.433417202922,-18.5927577129174));
#52679=CARTESIAN_POINT('Ctrl Pts',(16.2443944087803,-18.3496930245081,-18.5970112908029));
#52680=CARTESIAN_POINT('Ctrl Pts',(16.2659321081157,-18.2667421815311,-18.6012648686885));
#52681=CARTESIAN_POINT('Ctrl Pts',(16.2915956147072,-18.1850183713396,-18.605518446574));
#52682=CARTESIAN_POINT('Ctrl Pts',(16.3167615841415,-18.1048789366913,-18.6096895605515));
#52683=CARTESIAN_POINT('Ctrl Pts',(16.3458946705844,-18.0259198416596,-18.613860674529));
#52684=CARTESIAN_POINT('Ctrl Pts',(16.3788563531112,-17.9485567268056,-18.6180317885065));
#52685=CARTESIAN_POINT('Ctrl Pts',(16.411806975027,-17.8712195718919,-18.6222015028263));
#52686=CARTESIAN_POINT('Ctrl Pts',(16.4485834613785,-17.79547775642,-18.6263712171462));
#52687=CARTESIAN_POINT('Ctrl Pts',(16.4889988104968,-17.7217278109584,-18.6305409314661));
#52688=CARTESIAN_POINT('Ctrl Pts',(16.5294127214635,-17.6479804898363,-18.6347104974097));
#52689=CARTESIAN_POINT('Ctrl Pts',(16.5734650159172,-17.5762253008164,-18.6388800633533));
#52690=CARTESIAN_POINT('Ctrl Pts',(16.620922959331,-17.5068337741985,-18.6430496292968));
#52691=CARTESIAN_POINT('Ctrl Pts',(16.6700494655017,-17.4350025270905,-18.6473657920363));
#52692=CARTESIAN_POINT('Ctrl Pts',(16.7228252639786,-17.3657046830183,-18.6516819547758));
#52693=CARTESIAN_POINT('Ctrl Pts',(16.7789448088305,-17.2993175745228,-18.6559981175153));
#52694=CARTESIAN_POINT('Ctrl Pts',(16.8332362653982,-17.2350930191197,-18.6601736817066));
#52695=CARTESIAN_POINT('Ctrl Pts',(16.8906566126944,-17.1735927891267,-18.6643492458978));
#52696=CARTESIAN_POINT('Ctrl Pts',(16.9508909514351,-17.1151216368725,-18.668524810089));
#52697=CARTESIAN_POINT('Ctrl Pts',(17.0141675834549,-17.0536972456977,-18.6729112721026));
#52698=CARTESIAN_POINT('Ctrl Pts',(17.0805495076473,-16.9956163559342,-18.6772977341163));
#52699=CARTESIAN_POINT('Ctrl Pts',(17.1496333442479,-16.9411836731961,-18.6816841961299));
#52700=CARTESIAN_POINT('Ctrl Pts',(17.2187171808487,-16.886750990458,-18.6860706581436));
#52701=CARTESIAN_POINT('Ctrl Pts',(17.2905024122582,-16.835966787744,-18.6904571201572));
#52702=CARTESIAN_POINT('Ctrl Pts',(17.3645537444778,-16.7890813808106,-18.6948435821709));
#52703=CARTESIAN_POINT('Ctrl Pts',(17.4351978651041,-16.7443532409684,-18.6990282165633));
#52704=CARTESIAN_POINT('Ctrl Pts',(17.5081670866298,-16.703006515634,-18.7032128509558));
#52705=CARTESIAN_POINT('Ctrl Pts',(17.5831040926459,-16.665290877607,-18.7073974853483));
#52706=CARTESIAN_POINT('Ctrl Pts',(17.6579344351092,-16.6276289231224,-18.7115761634316));
#52707=CARTESIAN_POINT('Ctrl Pts',(17.734726591191,-16.5935879949174,-18.715754841515));
#52708=CARTESIAN_POINT('Ctrl Pts',(17.813095225772,-16.5633739520795,-18.7199335195984));
#52709=CARTESIAN_POINT('Ctrl Pts',(17.8928685618193,-16.532618344233,-18.7241870974839));
#52710=CARTESIAN_POINT('Ctrl Pts',(17.974275041662,-16.5058284229431,-18.7284406753695));
#52711=CARTESIAN_POINT('Ctrl Pts',(18.0568830023301,-16.4831718222066,-18.7326942532551));
#52712=CARTESIAN_POINT('Ctrl Pts',(18.13788944647,-16.4609544638901,-18.7368653672325));
#52713=CARTESIAN_POINT('Ctrl Pts',(18.2200507369796,-16.4427117186152,-18.7410364812098));
#52714=CARTESIAN_POINT('Ctrl Pts',(18.3029424071743,-16.428552090558,-18.7452075951871));
#52715=CARTESIAN_POINT('Ctrl Pts',(18.3858062622685,-16.4143972139007,-18.7493773095069));
#52716=CARTESIAN_POINT('Ctrl Pts',(18.4693995572162,-16.4043228107592,-18.7535470238267));
#52717=CARTESIAN_POINT('Ctrl Pts',(18.5532876521047,-16.3983862767995,-18.7577167381465));
#52718=CARTESIAN_POINT('Ctrl Pts',(18.6371727618947,-16.3924499540871,-18.7618863040899));
#52719=CARTESIAN_POINT('Ctrl Pts',(18.7213521918228,-16.3906512394234,-18.7660558700333));
#52720=CARTESIAN_POINT('Ctrl Pts',(18.8053875689175,-16.3929955422071,-18.7702254359768));
#52721=CARTESIAN_POINT('Ctrl Pts',(18.8923775262289,-16.3954222677854,-18.7745415987164));
#52722=CARTESIAN_POINT('Ctrl Pts',(18.9792125852183,-16.4022887536939,-18.778857761456));
#52723=CARTESIAN_POINT('Ctrl Pts',(19.0654100827152,-16.4135423271059,-18.7831739241957));
#52724=CARTESIAN_POINT('Ctrl Pts',(19.1487997057717,-16.4244293165444,-18.7873494883867));
#52725=CARTESIAN_POINT('Ctrl Pts',(19.2315922114996,-16.4394218336012,-18.7915250525778));
#52726=CARTESIAN_POINT('Ctrl Pts',(19.3133609024086,-16.4584200544678,-18.7957006167689));
#52727=CARTESIAN_POINT('Ctrl Pts',(19.3992595355481,-16.4783778303156,-18.8000870787828));
#52728=CARTESIAN_POINT('Ctrl Pts',(19.4840276488776,-16.5027564393573,-18.8044735407967));
#52729=CARTESIAN_POINT('Ctrl Pts',(19.5671906913809,-16.5313816344173,-18.8088600028106));
#52730=CARTESIAN_POINT('Ctrl Pts',(19.6503537338842,-16.5600068294773,-18.8132464648245));
#52731=CARTESIAN_POINT('Ctrl Pts',(19.7319111958456,-16.5928783231054,-18.8176329268384));
#52732=CARTESIAN_POINT('Ctrl Pts',(19.8114169849416,-16.6297655931066,-18.8220193888523));
#52733=CARTESIAN_POINT('Ctrl Pts',(19.8872706217461,-16.6649584213673,-18.8262043557615));
#52734=CARTESIAN_POINT('Ctrl Pts',(19.9615393050001,-16.7039371893188,-18.8303893226708));
#52735=CARTESIAN_POINT('Ctrl Pts',(20.0338195953306,-16.7465365521971,-18.83457428958));
#52736=CARTESIAN_POINT('Ctrl Pts',(20.1059885648684,-16.7890703066665,-18.8387528111107));
#52737=CARTESIAN_POINT('Ctrl Pts',(20.1761748342821,-16.8352133429708,-18.8429313326414));
#52738=CARTESIAN_POINT('Ctrl Pts',(20.2439967783581,-16.884753103921,-18.8471098541721));
#52739=CARTESIAN_POINT('Ctrl Pts',(20.2606541312307,-16.8969202762222,-18.8481361165208));
#52740=CARTESIAN_POINT('Ctrl Pts',(20.2771689760538,-16.9092921241003,-18.8491623788695));
#52741=CARTESIAN_POINT('Ctrl Pts',(20.293535888361,-16.9218650751948,-18.8501886412182));
#52742=CARTESIAN_POINT('Ctrl Pts',(20.293535888361,-16.9218650751948,-18.0500683203253));
#52743=CARTESIAN_POINT('Ctrl Pts',(20.3406388678367,-16.9580492647496,-18.0530337298048));
#52744=CARTESIAN_POINT('Ctrl Pts',(20.3864285999648,-16.9958326961473,-18.0559991392842));
#52745=CARTESIAN_POINT('Ctrl Pts',(20.43079571541,-17.0351055584184,-18.0589645487637));
#52746=CARTESIAN_POINT('Ctrl Pts',(20.4934043225857,-17.0905254157142,-18.0631491831568));
#52747=CARTESIAN_POINT('Ctrl Pts',(20.5534114448282,-17.1491189671381,-18.0673338175499));
#52748=CARTESIAN_POINT('Ctrl Pts',(20.6104778947947,-17.210612418114,-18.071518451943));
#52749=CARTESIAN_POINT('Ctrl Pts',(20.6674631177332,-17.2720183407738,-18.075697130027));
#52750=CARTESIAN_POINT('Ctrl Pts',(20.721515672228,-17.3363156298581,-18.079875808111));
#52751=CARTESIAN_POINT('Ctrl Pts',(20.7723306651571,-17.4031913935285,-18.084054486195));
#52752=CARTESIAN_POINT('Ctrl Pts',(20.8240564803135,-17.4712658571988,-18.0883080640805));
#52753=CARTESIAN_POINT('Ctrl Pts',(20.8724271646772,-17.5420118234209,-18.0925616419659));
#52754=CARTESIAN_POINT('Ctrl Pts',(20.9171616597699,-17.6150612701733,-18.0968152198513));
#52755=CARTESIAN_POINT('Ctrl Pts',(20.9610288893839,-17.6866945108573,-18.1009863338293));
#52756=CARTESIAN_POINT('Ctrl Pts',(21.0013994094996,-17.7605423037904,-18.1051574478073));
#52757=CARTESIAN_POINT('Ctrl Pts',(21.0380509604127,-17.8362270966629,-18.1093285617853));
#52758=CARTESIAN_POINT('Ctrl Pts',(21.0746902125439,-17.9118864927723,-18.1134982761058));
#52759=CARTESIAN_POINT('Ctrl Pts',(21.1076127735552,-17.9893812509009,-18.1176679904262));
#52760=CARTESIAN_POINT('Ctrl Pts',(21.136642647489,-18.068309834576,-18.1218377047466));
#52761=CARTESIAN_POINT('Ctrl Pts',(21.1656714884152,-18.1472356096333,-18.1260072706907));
#52762=CARTESIAN_POINT('Ctrl Pts',(21.1908077596747,-18.2275946767429,-18.1301768366348));
#52763=CARTESIAN_POINT('Ctrl Pts',(21.2119243630671,-18.3089674573408,-18.1343464025789));
#52764=CARTESIAN_POINT('Ctrl Pts',(21.2337834001839,-18.3932012045179,-18.1386625653178));
#52765=CARTESIAN_POINT('Ctrl Pts',(21.2513347146948,-18.478520765314,-18.1429787280566));
#52766=CARTESIAN_POINT('Ctrl Pts',(21.264494683606,-18.5644478664209,-18.1472948907955));
#52767=CARTESIAN_POINT('Ctrl Pts',(21.2772259679145,-18.6475759012496,-18.1514704549872));
#52768=CARTESIAN_POINT('Ctrl Pts',(21.2858476079666,-18.731272029579,-18.1556460191789));
#52769=CARTESIAN_POINT('Ctrl Pts',(21.290336834896,-18.8150986247191,-18.1598215833707));
#52770=CARTESIAN_POINT('Ctrl Pts',(21.2950528020053,-18.9031591018971,-18.1642080453831));
#52771=CARTESIAN_POINT('Ctrl Pts',(21.295207927637,-18.9913629881317,-18.1685945073955));
#52772=CARTESIAN_POINT('Ctrl Pts',(21.2908376238656,-19.0792059950831,-18.1729809694079));
#52773=CARTESIAN_POINT('Ctrl Pts',(21.2864673200943,-19.1670490020345,-18.1773674314203));
#52774=CARTESIAN_POINT('Ctrl Pts',(21.2775717212915,-19.2545305601574,-18.1817538934327));
#52775=CARTESIAN_POINT('Ctrl Pts',(21.2642482087235,-19.3411580684654,-18.1861403554451));
#52776=CARTESIAN_POINT('Ctrl Pts',(21.2515377307187,-19.4237997167046,-18.1903249898381));
#52777=CARTESIAN_POINT('Ctrl Pts',(21.2347505437471,-19.5059717882466,-18.1945096242311));
#52778=CARTESIAN_POINT('Ctrl Pts',(21.2139332700428,-19.5872408804027,-18.1986942586241));
#52779=CARTESIAN_POINT('Ctrl Pts',(21.193145627151,-19.6683942960652,-18.202872936708));
#52780=CARTESIAN_POINT('Ctrl Pts',(21.168339404859,-19.748646843478,-18.2070516147919));
#52781=CARTESIAN_POINT('Ctrl Pts',(21.1396126628223,-19.8275727933582,-18.2112302928758));
#52782=CARTESIAN_POINT('Ctrl Pts',(21.1103710145797,-19.9079134341683,-18.2154838707612));
#52783=CARTESIAN_POINT('Ctrl Pts',(21.0770669868023,-19.986878974605,-18.2197374486467));
#52784=CARTESIAN_POINT('Ctrl Pts',(21.039857896146,-20.0640338856263,-18.2239910265321));
#52785=CARTESIAN_POINT('Ctrl Pts',(21.0033701763203,-20.1396929981408,-18.22816214051));
#52786=CARTESIAN_POINT('Ctrl Pts',(20.9631276659828,-20.2136106264638,-18.2323332544879));
#52787=CARTESIAN_POINT('Ctrl Pts',(20.9193275219143,-20.2853955234528,-18.2365043684658));
#52788=CARTESIAN_POINT('Ctrl Pts',(20.8755420754071,-20.3571563323264,-18.2406740827861));
#52789=CARTESIAN_POINT('Ctrl Pts',(20.8282016054836,-20.4267854387981,-18.2448437971064));
#52790=CARTESIAN_POINT('Ctrl Pts',(20.7775484774992,-20.4939175140424,-18.2490135114267));
#52791=CARTESIAN_POINT('Ctrl Pts',(20.7268971519705,-20.5610472004393,-18.2531830773707));
#52792=CARTESIAN_POINT('Ctrl Pts',(20.672933680517,-20.6256796655625,-18.2573526433147));
#52793=CARTESIAN_POINT('Ctrl Pts',(20.6159420664663,-20.6874809300205,-18.2615222092587));
#52794=CARTESIAN_POINT('Ctrl Pts',(20.5569466975706,-20.7514550506984,-18.2658383719977));
#52795=CARTESIAN_POINT('Ctrl Pts',(20.4947066427107,-20.8123947886944,-18.2701545347367));
#52796=CARTESIAN_POINT('Ctrl Pts',(20.4295787905098,-20.8699709500337,-18.2744706974756));
#52797=CARTESIAN_POINT('Ctrl Pts',(20.3665724712459,-20.9256715739718,-18.2786462616673));
#52798=CARTESIAN_POINT('Ctrl Pts',(20.3008640027604,-20.9782241356929,-18.2828218258589));
#52799=CARTESIAN_POINT('Ctrl Pts',(20.2328090354881,-21.0273726111567,-18.2869973900505));
#52800=CARTESIAN_POINT('Ctrl Pts',(20.1613167736014,-21.0790034592787,-18.2913838520632));
#52801=CARTESIAN_POINT('Ctrl Pts',(20.0872352304043,-21.1268769860889,-18.2957703140758));
#52802=CARTESIAN_POINT('Ctrl Pts',(20.0110076004693,-21.1707500058239,-18.3001567760885));
#52803=CARTESIAN_POINT('Ctrl Pts',(19.9347799705344,-21.214623025559,-18.3045432381012));
#52804=CARTESIAN_POINT('Ctrl Pts',(19.8564068054921,-21.2544953429201,-18.3089297001138));
#52805=CARTESIAN_POINT('Ctrl Pts',(19.7763550154486,-21.2901822045703,-18.3133161621265));
#52806=CARTESIAN_POINT('Ctrl Pts',(19.6999865269343,-21.3242270608135,-18.3175007965194));
#52807=CARTESIAN_POINT('Ctrl Pts',(19.6218062328675,-21.3545898770089,-18.3216854309123));
#52808=CARTESIAN_POINT('Ctrl Pts',(19.5422037920528,-21.3810752624222,-18.3258700653053));
#52809=CARTESIAN_POINT('Ctrl Pts',(19.4627146554599,-21.4075229491676,-18.3300487433891));
#52810=CARTESIAN_POINT('Ctrl Pts',(19.3818078256885,-21.4301040236941,-18.3342274214729));
#52811=CARTESIAN_POINT('Ctrl Pts',(19.2998943515241,-21.4486704994679,-18.3384060995568));
#52812=CARTESIAN_POINT('Ctrl Pts',(19.2165126372027,-21.467569765977,-18.3426596774422));
#52813=CARTESIAN_POINT('Ctrl Pts',(19.1320882756879,-21.4823088984316,-18.3469132553277));
#52814=CARTESIAN_POINT('Ctrl Pts',(19.0470726305021,-21.4927844316334,-18.3511668332132));
#52815=CARTESIAN_POINT('Ctrl Pts',(18.9637051794954,-21.5030568761824,-18.355337947191));
#52816=CARTESIAN_POINT('Ctrl Pts',(18.8797696442091,-21.5092295037566,-18.3595090611688));
#52817=CARTESIAN_POINT('Ctrl Pts',(18.7957017187999,-21.5112563173502,-18.3636801751467));
#52818=CARTESIAN_POINT('Ctrl Pts',(18.7116620031949,-21.513282450827,-18.3678498894669));
#52819=CARTESIAN_POINT('Ctrl Pts',(18.6274904452119,-21.5111655221263,-18.3720196037872));
#52820=CARTESIAN_POINT('Ctrl Pts',(18.5436254163484,-21.5049115765924,-18.3761893181075));
#52821=CARTESIAN_POINT('Ctrl Pts',(18.4597633717625,-21.4986578536007,-18.3803588840514));
#52822=CARTESIAN_POINT('Ctrl Pts',(18.3762082933047,-21.4882674415331,-18.3845284499953));
#52823=CARTESIAN_POINT('Ctrl Pts',(18.2933947304044,-21.4737983655329,-18.3886980159393));
#52824=CARTESIAN_POINT('Ctrl Pts',(18.2076695447891,-21.4588205746693,-18.3930141786783));
#52825=CARTESIAN_POINT('Ctrl Pts',(18.1227395078358,-21.4394720625982,-18.3973303414174));
#52826=CARTESIAN_POINT('Ctrl Pts',(18.0390745966241,-21.415874729718,-18.4016465041564));
#52827=CARTESIAN_POINT('Ctrl Pts',(17.9581350610998,-21.3930460774757,-18.405822068348));
#52828=CARTESIAN_POINT('Ctrl Pts',(17.878379925585,-21.3662413589922,-18.4099976325396));
#52829=CARTESIAN_POINT('Ctrl Pts',(17.8002169726158,-21.3356210390432,-18.4141731967311));
#52830=CARTESIAN_POINT('Ctrl Pts',(17.7181061946998,-21.3034541595236,-18.4185596587439));
#52831=CARTESIAN_POINT('Ctrl Pts',(17.6377532005344,-21.2670763374213,-18.4229461207567));
#52832=CARTESIAN_POINT('Ctrl Pts',(17.559602363678,-21.2267285973938,-18.4273325827695));
#52833=CARTESIAN_POINT('Ctrl Pts',(17.4814515268215,-21.1863808573663,-18.4317190447823));
#52834=CARTESIAN_POINT('Ctrl Pts',(17.4055033100765,-21.1420635575358,-18.4361055067951));
#52835=CARTESIAN_POINT('Ctrl Pts',(17.3321657913464,-21.0940692919344,-18.4404919688079));
#52836=CARTESIAN_POINT('Ctrl Pts',(17.2622960528831,-21.0483444454524,-18.4446710160258));
#52837=CARTESIAN_POINT('Ctrl Pts',(17.19453408493,-20.9991112651902,-18.4488500632436));
#52838=CARTESIAN_POINT('Ctrl Pts',(17.1292545139165,-20.9465906660001,-18.4530291104615));
#52839=CARTESIAN_POINT('Ctrl Pts',(17.0640679209105,-20.8941448721524,-18.4572022054423));
#52840=CARTESIAN_POINT('Ctrl Pts',(17.0013570587501,-20.8384212459578,-18.461375300423));
#52841=CARTESIAN_POINT('Ctrl Pts',(16.9414683281885,-20.7796843834625,-18.4655483954038));
#52842=CARTESIAN_POINT('Ctrl Pts',(16.8809773183908,-20.7203568256503,-18.4697634576868));
#52843=CARTESIAN_POINT('Ctrl Pts',(16.8233659292103,-20.6579553356915,-18.4739785199699));
#52844=CARTESIAN_POINT('Ctrl Pts',(16.7689574885196,-20.5927949073772,-18.4781935822529));
#52845=CARTESIAN_POINT('Ctrl Pts',(16.715187711247,-20.5283993526991,-18.4823591668069));
#52846=CARTESIAN_POINT('Ctrl Pts',(16.6645463875622,-20.4613096522779,-18.4865247513609));
#52847=CARTESIAN_POINT('Ctrl Pts',(16.6173078768047,-20.3918661241945,-18.4906903359149));
#52848=CARTESIAN_POINT('Ctrl Pts',(16.5700850499656,-20.3224456524398,-18.4948545374302));
#52849=CARTESIAN_POINT('Ctrl Pts',(16.5262630517185,-20.2506732862345,-18.4990187389455));
#52850=CARTESIAN_POINT('Ctrl Pts',(16.4860739671284,-20.1769198140034,-18.5031829404608));
#52851=CARTESIAN_POINT('Ctrl Pts',(16.4458860826634,-20.1031685441962,-18.5073470176248));
#52852=CARTESIAN_POINT('Ctrl Pts',(16.4093311160888,-20.0274366916313,-18.5115110947889));
#52853=CARTESIAN_POINT('Ctrl Pts',(16.3765953977372,-19.9501200034215,-18.5156751719529));
#52854=CARTESIAN_POINT('Ctrl Pts',(16.3431614559385,-19.8711542197504,-18.5199280651399));
#52855=CARTESIAN_POINT('Ctrl Pts',(16.313711777103,-19.7905356687049,-18.5241809583268));
#52856=CARTESIAN_POINT('Ctrl Pts',(16.2883925214925,-19.7087060598861,-18.5284338515138));
#52857=CARTESIAN_POINT('Ctrl Pts',(16.2635663208297,-19.6284699613234,-18.5326039259141));
#52858=CARTESIAN_POINT('Ctrl Pts',(16.2427111716313,-19.5470700198228,-18.5367740003145));
#52859=CARTESIAN_POINT('Ctrl Pts',(16.2259135016087,-19.4649348073461,-18.5409440747148));
#52860=CARTESIAN_POINT('Ctrl Pts',(16.2086154222952,-19.3803527541242,-18.5452383772951));
#52861=CARTESIAN_POINT('Ctrl Pts',(16.1956204803925,-19.294991452669,-18.5495326798753));
#52862=CARTESIAN_POINT('Ctrl Pts',(16.1869656326132,-19.2093245642189,-18.5538269824556));
#52863=CARTESIAN_POINT('Ctrl Pts',(16.1783107848339,-19.1236576757689,-18.5581212850358));
#52864=CARTESIAN_POINT('Ctrl Pts',(16.1739959871027,-19.0376857298059,-18.5624155876161));
#52865=CARTESIAN_POINT('Ctrl Pts',(16.1740000028035,-18.9518801919504,-18.5667098901964));
#52866=CARTESIAN_POINT('Origin',(18.734,-18.952,1.76670989022851));
#52867=CARTESIAN_POINT('',(20.2917780564659,-16.9241894633619,-17.2500265416684));
#52868=CARTESIAN_POINT('',(20.294455276885,-16.9206896363573,-17.3168007021646));
#52869=CARTESIAN_POINT('',(20.293535888361,-16.9218650751948,1.76670989022851));
#52870=CARTESIAN_POINT('',(16.1740010840393,-18.9543559031924,-17.8332901097715));
#52871=CARTESIAN_POINT('Ctrl Pts',(20.294455276885,-16.9206896363574,-17.3168007021646));
#52872=CARTESIAN_POINT('Ctrl Pts',(20.846620702996,-17.3535718202006,-17.3517574545992));
#52873=CARTESIAN_POINT('Ctrl Pts',(21.6812137686398,-18.8317283057607,-17.4291061425942));
#52874=CARTESIAN_POINT('Ctrl Pts',(20.5976437703141,-21.3373977591934,-17.5488467661498));
#52875=CARTESIAN_POINT('Ctrl Pts',(17.7370130079676,-21.8102000472194,-17.6760225728312));
#52876=CARTESIAN_POINT('Ctrl Pts',(16.2862274700061,-20.2077259602722,-17.7708370079896));
#52877=CARTESIAN_POINT('Ctrl Pts',(16.1722336653236,-19.1559927438033,-17.8232595075876));
#52878=CARTESIAN_POINT('Ctrl Pts',(16.1740883619038,-18.9543565896946,-17.833290071625));
#52879=CARTESIAN_POINT('Ctrl Pts',(16.1740010840393,-18.9543559031924,-17.8332901097715));
#52880=CARTESIAN_POINT('Ctrl Pts',(16.1739248258781,-18.8714913735434,-17.837412174938));
#52881=CARTESIAN_POINT('Ctrl Pts',(16.177876160498,-18.7885152466554,-17.8415342401044));
#52882=CARTESIAN_POINT('Ctrl Pts',(16.1858608731257,-18.7058557534858,-17.8456563052709));
#52883=CARTESIAN_POINT('Ctrl Pts',(16.1938402258665,-18.6232517470386,-17.8497756034244));
#52884=CARTESIAN_POINT('Ctrl Pts',(16.205847540348,-18.5409644216311,-17.853894901578));
#52885=CARTESIAN_POINT('Ctrl Pts',(16.2218365582967,-18.4594202174575,-17.8580141997315));
#52886=CARTESIAN_POINT('Ctrl Pts',(16.2378199266111,-18.3779048264942,-17.862132042353));
#52887=CARTESIAN_POINT('Ctrl Pts',(16.2577821151893,-18.2971324990612,-17.8662498849744));
#52888=CARTESIAN_POINT('Ctrl Pts',(16.2816254461127,-18.2175212409839,-17.8703677275959));
#52889=CARTESIAN_POINT('Ctrl Pts',(16.3054679320359,-18.1379128043045,-17.8744854242824));
#52890=CARTESIAN_POINT('Ctrl Pts',(16.3331911499574,-18.0594658076281,-17.8786031209688));
#52891=CARTESIAN_POINT('Ctrl Pts',(16.364647494651,-17.9825833169392,-17.8827208176552));
#52892=CARTESIAN_POINT('Ctrl Pts',(16.396133878009,-17.905627408714,-17.8868424464612));
#52893=CARTESIAN_POINT('Ctrl Pts',(16.4313603282317,-17.8302394286303,-17.8909640752672));
#52894=CARTESIAN_POINT('Ctrl Pts',(16.470131238009,-17.7568020128526,-17.8950857040732));
#52895=CARTESIAN_POINT('Ctrl Pts',(16.5089205032735,-17.683329829267,-17.8992092842006));
#52896=CARTESIAN_POINT('Ctrl Pts',(16.5512573267501,-17.6118104548626,-17.903332864328));
#52897=CARTESIAN_POINT('Ctrl Pts',(16.5969016205558,-17.5425992349311,-17.9074564444553));
#52898=CARTESIAN_POINT('Ctrl Pts',(16.6426258760308,-17.4732667677586,-17.9115872484506));
#52899=CARTESIAN_POINT('Ctrl Pts',(16.691668894117,-17.4062509123682,-17.915718052446));
#52900=CARTESIAN_POINT('Ctrl Pts',(16.743749207993,-17.3418752269108,-17.9198488564413));
#52901=CARTESIAN_POINT('Ctrl Pts',(16.7879829276106,-17.2871985975131,-17.9233572996922));
#52902=CARTESIAN_POINT('Ctrl Pts',(16.8344068718464,-17.2344260450368,-17.9268657429432));
#52903=CARTESIAN_POINT('Ctrl Pts',(16.8828286089277,-17.1837340469049,-17.9303741861941));
#52904=CARTESIAN_POINT('Ctrl Pts',(16.9405827898754,-17.1232720517519,-17.9345588205871));
#52905=CARTESIAN_POINT('Ctrl Pts',(17.0014097311533,-17.0655300202436,-17.9387434549801));
#52906=CARTESIAN_POINT('Ctrl Pts',(17.0650229727702,-17.0108365131759,-17.9429280893731));
#52907=CARTESIAN_POINT('Ctrl Pts',(17.1285456688113,-16.9562208555459,-17.947106767457));
#52908=CARTESIAN_POINT('Ctrl Pts',(17.1948464417151,-16.9046454006959,-17.9512854455408));
#52909=CARTESIAN_POINT('Ctrl Pts',(17.2636010628229,-16.8564029572581,-17.9554641236247));
#52910=CARTESIAN_POINT('Ctrl Pts',(17.3335880611023,-16.807295802692,-17.9597177015102));
#52911=CARTESIAN_POINT('Ctrl Pts',(17.4061174102896,-16.7616426719217,-17.9639712793956));
#52912=CARTESIAN_POINT('Ctrl Pts',(17.4808106950308,-16.7197104654837,-17.9682248572811));
#52913=CARTESIAN_POINT('Ctrl Pts',(17.5540559046941,-16.6785911966922,-17.972395971259));
#52914=CARTESIAN_POINT('Ctrl Pts',(17.6293814748141,-16.6410501005274,-17.9765670852369));
#52915=CARTESIAN_POINT('Ctrl Pts',(17.7064016963159,-16.6072949596451,-17.9807381992148));
#52916=CARTESIAN_POINT('Ctrl Pts',(17.7833960729384,-16.5735511456264,-17.9849079135351));
#52917=CARTESIAN_POINT('Ctrl Pts',(17.8620835505878,-16.5435909483342,-17.9890776278554));
#52918=CARTESIAN_POINT('Ctrl Pts',(17.942056207647,-16.5175750104483,-17.9932473421757));
#52919=CARTESIAN_POINT('Ctrl Pts',(18.0220260189362,-16.4915599983211,-17.9974169081197));
#52920=CARTESIAN_POINT('Ctrl Pts',(18.1032804809772,-16.4694891080432,-18.0015864740637));
#52921=CARTESIAN_POINT('Ctrl Pts',(18.185395497294,-16.4514734355319,-18.0057560400077));
#52922=CARTESIAN_POINT('Ctrl Pts',(18.270397576287,-16.4328243541994,-18.0100722027467));
#52923=CARTESIAN_POINT('Ctrl Pts',(18.3563213344852,-16.4185210722996,-18.0143883654857));
#52924=CARTESIAN_POINT('Ctrl Pts',(18.4426856715113,-16.4086290160464,-18.0187045282247));
#52925=CARTESIAN_POINT('Ctrl Pts',(18.5262366993404,-16.3990591924854,-18.0228800924163));
#52926=CARTESIAN_POINT('Ctrl Pts',(18.6101995699748,-16.3936175999792,-18.0270556566079));
#52927=CARTESIAN_POINT('Ctrl Pts',(18.6941361080731,-16.3923103957471,-18.0312312207995));
#52928=CARTESIAN_POINT('Ctrl Pts',(18.7823120811743,-16.3909371677368,-18.0356176828122));
#52929=CARTESIAN_POINT('Ctrl Pts',(18.870458408217,-16.3941269389876,-18.0400041448249));
#52930=CARTESIAN_POINT('Ctrl Pts',(18.9580725064405,-16.4018251997446,-18.0443906068375));
#52931=CARTESIAN_POINT('Ctrl Pts',(19.0456866046639,-16.4095234605017,-18.0487770688502));
#52932=CARTESIAN_POINT('Ctrl Pts',(19.132767910028,-16.4217300548923,-18.0531635308629));
#52933=CARTESIAN_POINT('Ctrl Pts',(19.2188278686569,-16.4383289917386,-18.0575499928755));
#52934=CARTESIAN_POINT('Ctrl Pts',(19.3009320014006,-16.4541649430446,-18.06173482709));
#52935=CARTESIAN_POINT('Ctrl Pts',(19.3824122424308,-16.4740572520235,-18.0659196613044));
#52936=CARTESIAN_POINT('Ctrl Pts',(19.4628372070832,-16.4979428846151,-18.0701044955188));
#52937=CARTESIAN_POINT('Ctrl Pts',(19.5431287709651,-16.5217888981431,-18.0742823883549));
#52938=CARTESIAN_POINT('Ctrl Pts',(19.6223681012692,-16.5496149366889,-18.078460281191));
#52939=CARTESIAN_POINT('Ctrl Pts',(19.700133730563,-16.5813069336862,-18.0826381740271));
#52940=CARTESIAN_POINT('Ctrl Pts',(19.7778242916654,-16.6129683379793,-18.0868120338879));
#52941=CARTESIAN_POINT('Ctrl Pts',(19.8540435523397,-16.648488119696,-18.0909858937488));
#52942=CARTESIAN_POINT('Ctrl Pts',(19.9283857679273,-16.6877026172844,-18.0951597536096));
#52943=CARTESIAN_POINT('Ctrl Pts',(20.0026788000524,-16.726891171272,-18.0993308521204));
#52944=CARTESIAN_POINT('Ctrl Pts',(20.075096847298,-16.7697693732459,-18.1035019506312));
#52945=CARTESIAN_POINT('Ctrl Pts',(20.1452559587291,-16.8161262633405,-18.107673049142));
#52946=CARTESIAN_POINT('Ctrl Pts',(20.1959047159558,-16.8495918934532,-18.1106842183477));
#52947=CARTESIAN_POINT('Ctrl Pts',(20.2453766322748,-16.8848694611075,-18.1136953875534));
#52948=CARTESIAN_POINT('Ctrl Pts',(20.293535888361,-16.9218650751948,-18.1167065567592));
#52949=CARTESIAN_POINT('',(16.1740009581142,-18.9497851537726,-17.7667099127478));
#52950=CARTESIAN_POINT('Ctrl Pts',(16.1740009581142,-18.9497851537726,-17.7667099127478));
#52951=CARTESIAN_POINT('Ctrl Pts',(16.1740887027229,-18.8483667747388,-17.7717442924632));
#52952=CARTESIAN_POINT('Ctrl Pts',(16.1802070184517,-18.74721232135,-17.7767786721785));
#52953=CARTESIAN_POINT('Ctrl Pts',(16.1922394471764,-18.6469536230176,-17.7818130518939));
#52954=CARTESIAN_POINT('Ctrl Pts',(16.2044426849046,-18.5452716801573,-17.78691889826));
#52955=CARTESIAN_POINT('Ctrl Pts',(16.2227290670666,-18.4445110968517,-17.7920247446261));
#52956=CARTESIAN_POINT('Ctrl Pts',(16.2469282568539,-18.3453088558055,-17.7971305909922));
#52957=CARTESIAN_POINT('Ctrl Pts',(16.2587491290733,-18.2968503319625,-17.7996247057951));
#52958=CARTESIAN_POINT('Ctrl Pts',(16.2719801580747,-18.2487633198967,-17.8021188205979));
#52959=CARTESIAN_POINT('Ctrl Pts',(16.2865973915759,-18.201120201178,-17.8046129354008));
#52960=CARTESIAN_POINT('Ctrl Pts',(16.3111222362101,-18.1211844127561,-17.8087975697938));
#52961=CARTESIAN_POINT('Ctrl Pts',(16.3396130703746,-18.0423026572186,-17.8129822041869));
#52962=CARTESIAN_POINT('Ctrl Pts',(16.3719611025222,-17.9648970434642,-17.8171668385799));
#52963=CARTESIAN_POINT('Ctrl Pts',(16.4042630912499,-17.8876016070201,-17.8213455166639));
#52964=CARTESIAN_POINT('Ctrl Pts',(16.440411196743,-17.8117785597319,-17.8255241947478));
#52965=CARTESIAN_POINT('Ctrl Pts',(16.4802468398231,-17.7378349811527,-17.8297028728318));
#52966=CARTESIAN_POINT('Ctrl Pts',(16.5207965081759,-17.6625660170697,-17.8339564507172));
#52967=CARTESIAN_POINT('Ctrl Pts',(16.5651670712163,-17.5892450243182,-17.8382100286026));
#52968=CARTESIAN_POINT('Ctrl Pts',(16.6131398985284,-17.5182802121802,-17.8424636064881));
#52969=CARTESIAN_POINT('Ctrl Pts',(16.6601826789718,-17.448691191402,-17.846634720466));
#52970=CARTESIAN_POINT('Ctrl Pts',(16.7106890267627,-17.3813682068563,-17.8508058344439));
#52971=CARTESIAN_POINT('Ctrl Pts',(16.7644072919755,-17.3166698912768,-17.8549769484219));
#52972=CARTESIAN_POINT('Ctrl Pts',(16.8181075315056,-17.2519932858419,-17.8591466627423));
#52973=CARTESIAN_POINT('Ctrl Pts',(16.8750172543249,-17.1899399538654,-17.8633163770626));
#52974=CARTESIAN_POINT('Ctrl Pts',(16.9348438240379,-17.1308363460421,-17.867486091383));
#52975=CARTESIAN_POINT('Ctrl Pts',(16.9946682648647,-17.0717348413788,-17.871655657327));
#52976=CARTESIAN_POINT('Ctrl Pts',(17.0574090183535,-17.0155831748762,-17.8758252232711));
#52977=CARTESIAN_POINT('Ctrl Pts',(17.1227367799307,-16.9626707573527,-17.8799947892151));
#52978=CARTESIAN_POINT('Ctrl Pts',(17.1903613850146,-16.9078980045034,-17.884310951954));
#52979=CARTESIAN_POINT('Ctrl Pts',(17.2607578915086,-16.8565968547188,-17.8886271146929));
#52980=CARTESIAN_POINT('Ctrl Pts',(17.3335255671368,-16.8090414462952,-17.8929432774319));
#52981=CARTESIAN_POINT('Ctrl Pts',(17.403922843385,-16.7630351502993,-17.8971188416235));
#52982=CARTESIAN_POINT('Ctrl Pts',(17.4765387490618,-16.7205345053978,-17.9012944058152));
#52983=CARTESIAN_POINT('Ctrl Pts',(17.5509843556044,-16.681741427697,-17.9054699700069));
#52984=CARTESIAN_POINT('Ctrl Pts',(17.6291900327561,-16.6409890038631,-17.9098564320194));
#52985=CARTESIAN_POINT('Ctrl Pts',(17.7094145736833,-16.6043287713981,-17.914242894032));
#52986=CARTESIAN_POINT('Ctrl Pts',(17.7911842815274,-16.5719372863303,-17.9186293560446));
#52987=CARTESIAN_POINT('Ctrl Pts',(17.8729539893715,-16.5395458012624,-17.9230158180571));
#52988=CARTESIAN_POINT('Ctrl Pts',(17.9562682900625,-16.5114231770868,-17.9274022800697));
#52989=CARTESIAN_POINT('Ctrl Pts',(18.0406384682269,-16.4876847226345,-17.9317887420822));
#52990=CARTESIAN_POINT('Ctrl Pts',(18.1211305077812,-16.465037424071,-17.9359735770737));
#52991=CARTESIAN_POINT('Ctrl Pts',(18.2028831083918,-16.4462957978936,-17.9401584120651));
#52992=CARTESIAN_POINT('Ctrl Pts',(18.2854823965109,-16.4315968657057,-17.9443432470566));
#52993=CARTESIAN_POINT('Ctrl Pts',(18.3679630513099,-16.4169190448757,-17.9485220715741));
#52994=CARTESIAN_POINT('Ctrl Pts',(18.4512875288656,-16.406272464111,-17.9527008960917));
#52995=CARTESIAN_POINT('Ctrl Pts',(18.5350276579563,-16.3997441336924,-17.9568797206092));
#52996=CARTESIAN_POINT('Ctrl Pts',(18.6186666109273,-16.3932236909036,-17.9610534962063));
#52997=CARTESIAN_POINT('Ctrl Pts',(18.702719760757,-16.3908116415349,-17.9652272718033));
#52998=CARTESIAN_POINT('Ctrl Pts',(18.7867510727816,-16.3925435490479,-17.9694010474004));
#52999=CARTESIAN_POINT('Ctrl Pts',(18.8707269523644,-16.3942743140836,-17.9735720697075));
#53000=CARTESIAN_POINT('Ctrl Pts',(18.9546805641743,-16.4001435983918,-17.9777430920145));
#53001=CARTESIAN_POINT('Ctrl Pts',(19.0381741527013,-16.4101349200187,-17.9819141143216));
#53002=CARTESIAN_POINT('Ctrl Pts',(19.1216377101414,-16.4201226479535,-17.9860836363897));
#53003=CARTESIAN_POINT('Ctrl Pts',(19.20464111675,-16.4342294129592,-17.9902531584578));
#53004=CARTESIAN_POINT('Ctrl Pts',(19.2867513915057,-16.4523868500929,-17.994422680526));
#53005=CARTESIAN_POINT('Ctrl Pts',(19.3688567634641,-16.4705432030477,-17.9985919536323));
#53006=CARTESIAN_POINT('Ctrl Pts',(19.4500686609567,-16.4927496461544,-18.0027612267386));
#53007=CARTESIAN_POINT('Ctrl Pts',(19.5299652993024,-16.5188869236498,-18.0069304998449));
#53008=CARTESIAN_POINT('Ctrl Pts',(19.6099224331162,-16.5450439915502,-18.0111029298066));
#53009=CARTESIAN_POINT('Ctrl Pts',(19.6885618814584,-16.5751376935414,-18.0152753597682));
#53010=CARTESIAN_POINT('Ctrl Pts',(19.7654786756165,-16.6089994149065,-18.0194477897299));
#53011=CARTESIAN_POINT('Ctrl Pts',(19.8424284165325,-16.6428756406975,-18.023622006922));
#53012=CARTESIAN_POINT('Ctrl Pts',(19.9176536212663,-16.6805228962852,-18.0277962241141));
#53013=CARTESIAN_POINT('Ctrl Pts',(19.9907728936478,-16.7217260496091,-18.0319704413063));
#53014=CARTESIAN_POINT('Ctrl Pts',(20.0639908538905,-16.7629848141412,-18.0361502923696));
#53015=CARTESIAN_POINT('Ctrl Pts',(20.1350968176494,-16.807808813561,-18.040330143433));
#53016=CARTESIAN_POINT('Ctrl Pts',(20.2037378785288,-16.8559392736808,-18.0445099944964));
#53017=CARTESIAN_POINT('Ctrl Pts',(20.2341639531921,-16.8772737483295,-18.0463627697727));
#53018=CARTESIAN_POINT('Ctrl Pts',(20.2641061463923,-16.8992573468981,-18.048215545049));
#53019=CARTESIAN_POINT('Ctrl Pts',(20.293535888361,-16.9218650751948,-18.0500683203253));
#53020=CARTESIAN_POINT('Ctrl Pts',(20.2917780564658,-16.9241894633618,-17.2500265416684));
#53021=CARTESIAN_POINT('Ctrl Pts',(20.5375805774977,-17.1103101642375,-17.2653209306706));
#53022=CARTESIAN_POINT('Ctrl Pts',(21.3400060360654,-17.9709561757374,-17.3230072552333));
#53023=CARTESIAN_POINT('Ctrl Pts',(21.4691813208793,-20.2489483349579,-17.4230855153565));
#53024=CARTESIAN_POINT('Ctrl Pts',(19.1239734689994,-21.9538681741735,-17.5502613220379));
#53025=CARTESIAN_POINT('Ctrl Pts',(16.6895185822271,-21.0089844641567,-17.6648027803286));
#53026=CARTESIAN_POINT('Ctrl Pts',(16.1805386002103,-19.5488856395492,-17.7369523030588));
#53027=CARTESIAN_POINT('Ctrl Pts',(16.1756126004107,-18.9497870014945,-17.7667098902285));
#53028=CARTESIAN_POINT('Origin',(18.734,-18.952,1.76670989022851));
#53029=CARTESIAN_POINT('',(20.293535888361,-16.9218650751947,-16.4501666918036));
#53030=CARTESIAN_POINT('',(20.293535888361,-16.9218650751947,-16.516630357267));
#53031=CARTESIAN_POINT('',(20.293535888361,-16.9218650751948,1.76670989022851));
#53032=CARTESIAN_POINT('',(16.1737370593341,-18.9511644347003,-17.0332901097715));
#53033=CARTESIAN_POINT('Ctrl Pts',(20.293535888361,-16.9218650751947,-16.516630357267));
#53034=CARTESIAN_POINT('Ctrl Pts',(20.3601025931298,-16.9730011665887,-16.5208151876277));
#53035=CARTESIAN_POINT('Ctrl Pts',(20.4240566331923,-17.0273416960463,-16.5250000179883));
#53036=CARTESIAN_POINT('Ctrl Pts',(20.4850922791488,-17.0845750805172,-16.529184848349));
#53037=CARTESIAN_POINT('Ctrl Pts',(20.4960575761564,-17.0948572860978,-16.5299366697988));
#53038=CARTESIAN_POINT('Ctrl Pts',(20.506928783665,-17.1052327721162,-16.5306884912485));
#53039=CARTESIAN_POINT('Ctrl Pts',(20.5177042670234,-17.115699619397,-16.5314403126983));
#53040=CARTESIAN_POINT('Ctrl Pts',(20.5776805529838,-17.1739580385085,-16.5356249470914));
#53041=CARTESIAN_POINT('Ctrl Pts',(20.6349112416909,-17.2352663353223,-16.5398095814844));
#53042=CARTESIAN_POINT('Ctrl Pts',(20.6890701824651,-17.2993353087707,-16.5439942158775));
#53043=CARTESIAN_POINT('Ctrl Pts',(20.7431520346907,-17.3633130879657,-16.5481728939614));
#53044=CARTESIAN_POINT('Ctrl Pts',(20.7941705292093,-17.4300433902867,-16.5523515720453));
#53045=CARTESIAN_POINT('Ctrl Pts',(20.8418355824982,-17.4991995466842,-16.5565302501293));
#53046=CARTESIAN_POINT('Ctrl Pts',(20.8903549976109,-17.5695952774835,-16.5607838280147));
#53047=CARTESIAN_POINT('Ctrl Pts',(20.9353992222982,-17.6425043486949,-16.5650374059002));
#53048=CARTESIAN_POINT('Ctrl Pts',(20.9767045339426,-17.7175461234078,-16.5692909837856));
#53049=CARTESIAN_POINT('Ctrl Pts',(21.01720906152,-17.7911330668859,-16.5734620977636));
#53050=CARTESIAN_POINT('Ctrl Pts',(21.0541181225501,-17.8667703369927,-16.5776332117415));
#53051=CARTESIAN_POINT('Ctrl Pts',(21.0872271712958,-17.9440704983605,-16.5818043257195));
#53052=CARTESIAN_POINT('Ctrl Pts',(21.1203251099804,-18.0213447209125,-16.5859740400399));
#53053=CARTESIAN_POINT('Ctrl Pts',(21.149625387836,-18.1002803040063,-16.5901437543602));
#53054=CARTESIAN_POINT('Ctrl Pts',(21.1749707834402,-18.1804679952254,-16.5943134686806));
#53055=CARTESIAN_POINT('Ctrl Pts',(21.2003152771464,-18.2606528330223,-16.5984830346246));
#53056=CARTESIAN_POINT('Ctrl Pts',(21.2217050305799,-18.3420892514568,-16.6026526005687));
#53057=CARTESIAN_POINT('Ctrl Pts',(21.2390325027795,-18.4243522386871,-16.6068221665127));
#53058=CARTESIAN_POINT('Ctrl Pts',(21.2569691875259,-18.5095074910661,-16.6111383292517));
#53059=CARTESIAN_POINT('Ctrl Pts',(21.2705525077454,-18.5955480019175,-16.6154544919906));
#53060=CARTESIAN_POINT('Ctrl Pts',(21.2797210678871,-18.6819921399002,-16.6197706547295));
#53061=CARTESIAN_POINT('Ctrl Pts',(21.2885909631465,-18.7656203691804,-16.6239462189212));
#53062=CARTESIAN_POINT('Ctrl Pts',(21.2933293236125,-18.8496258601582,-16.6281217831129));
#53063=CARTESIAN_POINT('Ctrl Pts',(21.2939336612287,-18.9335704012973,-16.6322973473045));
#53064=CARTESIAN_POINT('Ctrl Pts',(21.2945685225012,-19.0217547816502,-16.6366838093171));
#53065=CARTESIAN_POINT('Ctrl Pts',(21.2906407927078,-19.1098713098954,-16.6410702713296));
#53066=CARTESIAN_POINT('Ctrl Pts',(21.2822091879386,-19.197417877314,-16.6454567333422));
#53067=CARTESIAN_POINT('Ctrl Pts',(21.2737775831694,-19.2849644447327,-16.6498431953547));
#53068=CARTESIAN_POINT('Ctrl Pts',(21.2608422640144,-19.3719404886095,-16.6542296573672));
#53069=CARTESIAN_POINT('Ctrl Pts',(21.2435233083642,-19.4578584434176,-16.6586161193798));
#53070=CARTESIAN_POINT('Ctrl Pts',(21.2270012235362,-19.5398231857641,-16.6628007537728));
#53071=CARTESIAN_POINT('Ctrl Pts',(21.2064285344955,-19.6211301562754,-16.6669853881659));
#53072=CARTESIAN_POINT('Ctrl Pts',(21.1818718743957,-19.7013485747917,-16.6711700225589));
#53073=CARTESIAN_POINT('Ctrl Pts',(21.1573501676621,-19.7814528123184,-16.6753487006429));
#53074=CARTESIAN_POINT('Ctrl Pts',(21.1288558871501,-19.8604711393629,-16.6795273787268));
#53075=CARTESIAN_POINT('Ctrl Pts',(21.0965066931248,-19.9379828218283,-16.6837060568108));
#53076=CARTESIAN_POINT('Ctrl Pts',(21.0635776630456,-20.0168838454952,-16.6879596346962));
#53077=CARTESIAN_POINT('Ctrl Pts',(21.0266542567594,-20.0942232074709,-16.6922132125816));
#53078=CARTESIAN_POINT('Ctrl Pts',(20.98591378162,-20.1695731272289,-16.6964667904671));
#53079=CARTESIAN_POINT('Ctrl Pts',(20.9459631400897,-20.243462241759,-16.700637904445));
#53080=CARTESIAN_POINT('Ctrl Pts',(20.9023423404873,-20.3154379408342,-16.704809018423));
#53081=CARTESIAN_POINT('Ctrl Pts',(20.8552664379161,-20.3851185224436,-16.7089801324009));
#53082=CARTESIAN_POINT('Ctrl Pts',(20.8082063321186,-20.4547757220608,-16.7131498467213));
#53083=CARTESIAN_POINT('Ctrl Pts',(20.7576936832431,-20.5221389528648,-16.7173195610417));
#53084=CARTESIAN_POINT('Ctrl Pts',(20.7039875068322,-20.5868544959491,-16.721489275362));
#53085=CARTESIAN_POINT('Ctrl Pts',(20.6502832415176,-20.6515677361767,-16.7256588413061));
#53086=CARTESIAN_POINT('Ctrl Pts',(20.5933859690516,-20.713633122547,-16.7298284072501));
#53087=CARTESIAN_POINT('Ctrl Pts',(20.5335948472511,-20.7727301792818,-16.7339979731942));
#53088=CARTESIAN_POINT('Ctrl Pts',(20.4717015433682,-20.8339050156273,-16.7383141359331));
#53089=CARTESIAN_POINT('Ctrl Pts',(20.406707483555,-20.8918985349615,-16.742630298672));
#53090=CARTESIAN_POINT('Ctrl Pts',(20.3389844113022,-20.9463984154318,-16.7469464614109));
#53091=CARTESIAN_POINT('Ctrl Pts',(20.2734674110048,-20.9991229680282,-16.7511220256026));
#53092=CARTESIAN_POINT('Ctrl Pts',(20.2053968718997,-21.0485777582944,-16.7552975897943));
#53093=CARTESIAN_POINT('Ctrl Pts',(20.1351399138028,-21.0945234985756,-16.759473153986));
#53094=CARTESIAN_POINT('Ctrl Pts',(20.0613344437724,-21.1427898489728,-16.7638596159985));
#53095=CARTESIAN_POINT('Ctrl Pts',(19.9851163826192,-21.1871830552703,-16.7682460780111));
#53096=CARTESIAN_POINT('Ctrl Pts',(19.9069397062211,-21.2274807064816,-16.7726325400236));
#53097=CARTESIAN_POINT('Ctrl Pts',(19.828763029823,-21.2677783576928,-16.7770190020362));
#53098=CARTESIAN_POINT('Ctrl Pts',(19.748628298259,-21.3039802842616,-16.7814054640487));
#53099=CARTESIAN_POINT('Ctrl Pts',(19.6670104728628,-21.3359235427187,-16.7857919260613));
#53100=CARTESIAN_POINT('Ctrl Pts',(19.5891480045999,-21.3663970445028,-16.7899765604543));
#53101=CARTESIAN_POINT('Ctrl Pts',(19.5096461031211,-21.3931085897472,-16.7941611948473));
#53102=CARTESIAN_POINT('Ctrl Pts',(19.4289030536307,-21.4158810332593,-16.7983458292404));
#53103=CARTESIAN_POINT('Ctrl Pts',(19.3482749318772,-21.4386210630167,-16.8025245073243));
#53104=CARTESIAN_POINT('Ctrl Pts',(19.2664096101498,-21.4574330041518,-16.8067031854083));
#53105=CARTESIAN_POINT('Ctrl Pts',(19.1837245465112,-21.4721880549406,-16.8108818634922));
#53106=CARTESIAN_POINT('Ctrl Pts',(19.0995574125316,-21.4872075794106,-16.8151354413777));
#53107=CARTESIAN_POINT('Ctrl Pts',(19.0145413088146,-21.49802316776,-16.8193890192631));
#53108=CARTESIAN_POINT('Ctrl Pts',(18.9291319041929,-21.5045523579284,-16.8236425971485));
#53109=CARTESIAN_POINT('Ctrl Pts',(18.8453783275425,-21.5109549670048,-16.8278137111265));
#53110=CARTESIAN_POINT('Ctrl Pts',(18.7612470435307,-21.5132358584627,-16.8319848251044));
#53111=CARTESIAN_POINT('Ctrl Pts',(18.6771754083916,-21.5113692515517,-16.8361559390824));
#53112=CARTESIAN_POINT('Ctrl Pts',(18.5931319843017,-21.5095032709988,-16.8403256534027));
#53113=CARTESIAN_POINT('Ctrl Pts',(18.5091486288698,-21.5034925662839,-16.8444953677231));
#53114=CARTESIAN_POINT('Ctrl Pts',(18.4256629639196,-21.4933634671532,-16.8486650820435));
#53115=CARTESIAN_POINT('Ctrl Pts',(18.3421802697477,-21.4832347284594,-16.8528346479875));
#53116=CARTESIAN_POINT('Ctrl Pts',(18.2591956874268,-21.4689879429832,-16.8570042139316));
#53117=CARTESIAN_POINT('Ctrl Pts',(18.1771406148225,-21.4507011876452,-16.8611737798756));
#53118=CARTESIAN_POINT('Ctrl Pts',(18.0922005870914,-21.4317714925488,-16.8654899426145));
#53119=CARTESIAN_POINT('Ctrl Pts',(18.0082571631379,-21.4085125658604,-16.8698061053535));
#53120=CARTESIAN_POINT('Ctrl Pts',(17.9257741739147,-21.3810679311309,-16.8741222680924));
#53121=CARTESIAN_POINT('Ctrl Pts',(17.8459780593898,-21.3545173024911,-16.8782978322841));
#53122=CARTESIAN_POINT('Ctrl Pts',(17.7675491154084,-21.3240496914869,-16.8824733964757));
#53123=CARTESIAN_POINT('Ctrl Pts',(17.6908872600138,-21.2898442659165,-16.8866489606674));
#53124=CARTESIAN_POINT('Ctrl Pts',(17.6103533965495,-21.2539112056161,-16.8910354226799));
#53125=CARTESIAN_POINT('Ctrl Pts',(17.5317703445183,-21.2138530785411,-16.8954218846925));
#53126=CARTESIAN_POINT('Ctrl Pts',(17.4555708448951,-21.169931219713,-16.899808346705));
#53127=CARTESIAN_POINT('Ctrl Pts',(17.3793713452718,-21.1260093608849,-16.9041948087175));
#53128=CARTESIAN_POINT('Ctrl Pts',(17.3055558437865,-21.0782241494638,-16.9085812707301));
#53129=CARTESIAN_POINT('Ctrl Pts',(17.2345184376722,-21.0268867545577,-16.9129677327426));
#53130=CARTESIAN_POINT('Ctrl Pts',(17.167299168743,-20.9783086554537,-16.9171184300413));
#53131=CARTESIAN_POINT('Ctrl Pts',(17.1023079512147,-20.9263629083338,-16.9212691273401));
#53132=CARTESIAN_POINT('Ctrl Pts',(17.0399060592653,-20.8712826055498,-16.9254198246388));
#53133=CARTESIAN_POINT('Ctrl Pts',(16.9775932241692,-20.8162809106139,-16.9295645982704));
#53134=CARTESIAN_POINT('Ctrl Pts',(16.9178627255451,-20.7581538490648,-16.9337093719019));
#53135=CARTESIAN_POINT('Ctrl Pts',(16.8610458812396,-20.6971770308534,-16.9378541455334));
#53136=CARTESIAN_POINT('Ctrl Pts',(16.8042942087153,-20.6362701561228,-16.9419941649009));
#53137=CARTESIAN_POINT('Ctrl Pts',(16.7504498675423,-20.5725203603437,-16.9461341842684));
#53138=CARTESIAN_POINT('Ctrl Pts',(16.6998090154257,-20.506241628022,-16.9502742036359));
#53139=CARTESIAN_POINT('Ctrl Pts',(16.6491995836852,-20.4400040186794,-16.9544116543072));
#53140=CARTESIAN_POINT('Ctrl Pts',(16.6017899801564,-20.3712409577298,-16.9585491049784));
#53141=CARTESIAN_POINT('Ctrl Pts',(16.5578367768806,-20.3003002730633,-16.9626865556497));
#53142=CARTESIAN_POINT('Ctrl Pts',(16.5138971231855,-20.2293814574863,-16.9668227308571));
#53143=CARTESIAN_POINT('Ctrl Pts',(16.4734120005631,-20.1562867489274,-16.9709589060645));
#53144=CARTESIAN_POINT('Ctrl Pts',(16.4365944037611,-20.0813925475095,-16.9750950812719));
#53145=CARTESIAN_POINT('Ctrl Pts',(16.3997766632186,-20.0064980536954,-16.9792312726275));
#53146=CARTESIAN_POINT('Ctrl Pts',(16.366626681762,-19.9298044742117,-16.983367463983));
#53147=CARTESIAN_POINT('Ctrl Pts',(16.3373106052886,-19.8517110343203,-16.9875036553386));
#53148=CARTESIAN_POINT('Ctrl Pts',(16.3079666664254,-19.773543373383,-16.9916437777855));
#53149=CARTESIAN_POINT('Ctrl Pts',(16.2824640727847,-19.6939736349118,-16.9957839002324));
#53150=CARTESIAN_POINT('Ctrl Pts',(16.2609198329124,-19.6134185415892,-16.9999240226793));
#53151=CARTESIAN_POINT('Ctrl Pts',(16.2393648184702,-19.532823161559,-17.0040662156583));
#53152=CARTESIAN_POINT('Ctrl Pts',(16.2217721969233,-19.4512419037245,-17.0082084086373));
#53153=CARTESIAN_POINT('Ctrl Pts',(16.2082078057625,-19.3691016561093,-17.0123506016162));
#53154=CARTESIAN_POINT('Ctrl Pts',(16.1946210138151,-19.2868257587522,-17.016499635181));
#53155=CARTESIAN_POINT('Ctrl Pts',(16.1850757885661,-19.2039894937103,-17.0206486687457));
#53156=CARTESIAN_POINT('Ctrl Pts',(16.1795860271471,-19.1210244221821,-17.0247977023105));
#53157=CARTESIAN_POINT('Ctrl Pts',(16.1758404729028,-19.06441901585,-17.0276285047975));
#53158=CARTESIAN_POINT('Ctrl Pts',(16.1739816679355,-19.0077536994294,-17.0304593072845));
#53159=CARTESIAN_POINT('Ctrl Pts',(16.1740001363332,-18.9511645205579,-17.0332901097715));
#53160=CARTESIAN_POINT('Ctrl Pts',(16.1700998810729,-18.9511632476738,-17.0332901097715));
#53161=CARTESIAN_POINT('Ctrl Pts',(16.1699051733629,-18.905425756545,-17.0355745863224));
#53162=CARTESIAN_POINT('Ctrl Pts',(16.1917620149477,-18.0111494804083,-17.0802509984337));
#53163=CARTESIAN_POINT('Ctrl Pts',(17.2348044654712,-16.3222275152694,-17.1673193461055));
#53164=CARTESIAN_POINT('Ctrl Pts',(19.3369083681933,-16.2828821706046,-17.2595384003524));
#53165=CARTESIAN_POINT('Ctrl Pts',(20.177011556488,-16.8286170585391,-17.3093655190387));
#53166=CARTESIAN_POINT('Ctrl Pts',(20.294455276885,-16.9206896363574,-17.3168007021646));
#53167=CARTESIAN_POINT('',(16.1741505163153,-18.9531967450726,-16.9667098397546));
#53168=CARTESIAN_POINT('Ctrl Pts',(16.1776746515055,-18.9531940792248,-16.9667098902285));
#53169=CARTESIAN_POINT('Ctrl Pts',(16.1797896608842,-18.4498774694967,-16.9916592919231));
#53170=CARTESIAN_POINT('Ctrl Pts',(16.5671404047359,-17.0883638912152,-17.0590006291781));
#53171=CARTESIAN_POINT('Ctrl Pts',(18.4733994257987,-16.0873963198054,-17.1534395129914));
#53172=CARTESIAN_POINT('Ctrl Pts',(19.8562820548392,-16.5944336060539,-17.2229289951101));
#53173=CARTESIAN_POINT('Ctrl Pts',(20.2917780564658,-16.9241894633618,-17.2500265416684));
#53174=CARTESIAN_POINT('Ctrl Pts',(20.293535888361,-16.9218650751947,-16.4501666918036));
#53175=CARTESIAN_POINT('Ctrl Pts',(20.3601794064216,-16.9730601740388,-16.4543369075911));
#53176=CARTESIAN_POINT('Ctrl Pts',(20.4243360771708,-17.0275684722783,-16.4585071233785));
#53177=CARTESIAN_POINT('Ctrl Pts',(20.4856660020915,-17.0851132286299,-16.462677339166));
#53178=CARTESIAN_POINT('Ctrl Pts',(20.5469851039405,-17.1426478298895,-16.4668468190233));
#53179=CARTESIAN_POINT('Ctrl Pts',(20.6054781157674,-17.2032175098257,-16.4710162988806));
#53180=CARTESIAN_POINT('Ctrl Pts',(20.6608402898758,-17.2665070461995,-16.4751857787379));
#53181=CARTESIAN_POINT('Ctrl Pts',(20.7162093011933,-17.3298043988087,-16.4793557735244));
#53182=CARTESIAN_POINT('Ctrl Pts',(20.7684464051496,-17.3958219277228,-16.483525768311));
#53183=CARTESIAN_POINT('Ctrl Pts',(20.817286518905,-17.4642106062521,-16.4876957630976));
#53184=CARTESIAN_POINT('Ctrl Pts',(20.8661791251708,-17.5326727877516,-16.4918702397225));
#53185=CARTESIAN_POINT('Ctrl Pts',(20.9116671848706,-17.6035108313142,-16.4960447163474));
#53186=CARTESIAN_POINT('Ctrl Pts',(20.9535287399399,-17.6763463743709,-16.5002191929724));
#53187=CARTESIAN_POINT('Ctrl Pts',(20.9954147215154,-17.7492244174694,-16.5043961054332));
#53188=CARTESIAN_POINT('Ctrl Pts',(21.0336697764926,-17.8241018708103,-16.508573017894));
#53189=CARTESIAN_POINT('Ctrl Pts',(21.0681188608709,-17.9005775619065,-16.5127499303549));
#53190=CARTESIAN_POINT('Ctrl Pts',(21.1026261840292,-17.9771825409365,-16.5169339042018));
#53191=CARTESIAN_POINT('Ctrl Pts',(21.1333145214185,-18.0553907244829,-16.5211178780488));
#53192=CARTESIAN_POINT('Ctrl Pts',(21.1600578420673,-18.1347831701783,-16.5253018518957));
#53193=CARTESIAN_POINT('Ctrl Pts',(21.1761504177396,-18.1825569286034,-16.527819524126));
#53194=CARTESIAN_POINT('Ctrl Pts',(21.1908155027428,-18.2307592272839,-16.5303371963562));
#53195=CARTESIAN_POINT('Ctrl Pts',(21.2040345704695,-18.2792970784325,-16.5328548685865));
#53196=CARTESIAN_POINT('Ctrl Pts',(21.2260060426843,-18.3599720602032,-16.5370395029795));
#53197=CARTESIAN_POINT('Ctrl Pts',(21.244061800264,-18.4418747378537,-16.5412241373726));
#53198=CARTESIAN_POINT('Ctrl Pts',(21.2580683099057,-18.5245901651463,-16.5454087717656));
#53199=CARTESIAN_POINT('Ctrl Pts',(21.2720548830146,-18.607187857266,-16.5495874498496));
#53200=CARTESIAN_POINT('Ctrl Pts',(21.2820035803663,-18.6905955514662,-16.5537661279335));
#53201=CARTESIAN_POINT('Ctrl Pts',(21.28783098536,-18.7743844088622,-16.5579448060174));
#53202=CARTESIAN_POINT('Ctrl Pts',(21.2937628424001,-18.8596751213091,-16.5621983839029));
#53203=CARTESIAN_POINT('Ctrl Pts',(21.2954240788116,-18.9453603308623,-16.5664519617883));
#53204=CARTESIAN_POINT('Ctrl Pts',(21.2927814384536,-19.0309781629654,-16.5707055396738));
#53205=CARTESIAN_POINT('Ctrl Pts',(21.2901900308356,-19.1149361263238,-16.5748766536517));
#53206=CARTESIAN_POINT('Ctrl Pts',(21.2834601502021,-19.1988288204156,-16.5790477676297));
#53207=CARTESIAN_POINT('Ctrl Pts',(21.2726129381323,-19.2822186402178,-16.5832188816076));
#53208=CARTESIAN_POINT('Ctrl Pts',(21.2617693659493,-19.3655804777606,-16.587388595928));
#53209=CARTESIAN_POINT('Ctrl Pts',(21.246811265521,-19.4484393203326,-16.5915583102484));
#53210=CARTESIAN_POINT('Ctrl Pts',(21.2278116184524,-19.5303628719687,-16.5957280245688));
#53211=CARTESIAN_POINT('Ctrl Pts',(21.2088126474728,-19.6122835084131,-16.5998975905128));
#53212=CARTESIAN_POINT('Ctrl Pts',(21.1857725205575,-19.6932684721477,-16.6040671564568));
#53213=CARTESIAN_POINT('Ctrl Pts',(21.1588150040535,-19.7728971897365,-16.6082367224009));
#53214=CARTESIAN_POINT('Ctrl Pts',(21.1309096945249,-19.855325554803,-16.6125528851398));
#53215=CARTESIAN_POINT('Ctrl Pts',(21.0988065683011,-19.93630002845,-16.6168690478787));
#53216=CARTESIAN_POINT('Ctrl Pts',(21.0626979316573,-20.015374789571,-16.6211852106176));
#53217=CARTESIAN_POINT('Ctrl Pts',(21.0277655300541,-20.0918736986657,-16.6253607748093));
#53218=CARTESIAN_POINT('Ctrl Pts',(20.9890848280185,-20.1665943642433,-16.629536339001));
#53219=CARTESIAN_POINT('Ctrl Pts',(20.9468767362672,-20.239158323629,-16.6337119031927));
#53220=CARTESIAN_POINT('Ctrl Pts',(20.9025368141418,-20.3153873160988,-16.6380983652052));
#53221=CARTESIAN_POINT('Ctrl Pts',(20.8543041199709,-20.3892355173249,-16.6424848272177));
#53222=CARTESIAN_POINT('Ctrl Pts',(20.8024847707862,-20.4603006175911,-16.6468712892303));
#53223=CARTESIAN_POINT('Ctrl Pts',(20.7506654216015,-20.5313657178572,-16.6512577512428));
#53224=CARTESIAN_POINT('Ctrl Pts',(20.6952598420584,-20.5996473145404,-16.6556442132554));
#53225=CARTESIAN_POINT('Ctrl Pts',(20.6366195645772,-20.664786849695,-16.6600306752679));
#53226=CARTESIAN_POINT('Ctrl Pts',(20.5806774131886,-20.7269292182772,-16.664215309661));
#53227=CARTESIAN_POINT('Ctrl Pts',(20.5215834617877,-20.7864436190212,-16.668399944054));
#53228=CARTESIAN_POINT('Ctrl Pts',(20.4596143354494,-20.8429931690229,-16.6725845784471));
#53229=CARTESIAN_POINT('Ctrl Pts',(20.3977334144921,-20.8994622277398,-16.676763256531));
#53230=CARTESIAN_POINT('Ctrl Pts',(20.3329857844078,-20.9529745107158,-16.6809419346149));
#53231=CARTESIAN_POINT('Ctrl Pts',(20.2656868790094,-21.0032277554359,-16.6851206126989));
#53232=CARTESIAN_POINT('Ctrl Pts',(20.1971816890986,-21.0543817534511,-16.6893741905843));
#53233=CARTESIAN_POINT('Ctrl Pts',(20.1260331836046,-21.1021583691593,-16.6936277684698));
#53234=CARTESIAN_POINT('Ctrl Pts',(20.0526117250174,-21.1462796354719,-16.6978813463552));
#53235=CARTESIAN_POINT('Ctrl Pts',(19.980613684675,-21.1895455249415,-16.7020524603332));
#53236=CARTESIAN_POINT('Ctrl Pts',(19.9064304485057,-21.2292962845166,-16.7062235743111));
#53237=CARTESIAN_POINT('Ctrl Pts',(19.8304414166174,-21.2653128236203,-16.7103946882891));
#53238=CARTESIAN_POINT('Ctrl Pts',(19.7544778835828,-21.3013172770264,-16.7145644026094));
#53239=CARTESIAN_POINT('Ctrl Pts',(19.676710173617,-21.3335898016788,-16.7187341169298));
#53240=CARTESIAN_POINT('Ctrl Pts',(19.5975412827729,-21.3619577699509,-16.7229038312502));
#53241=CARTESIAN_POINT('Ctrl Pts',(19.5183752090976,-21.3903247287691,-16.7270733971942));
#53242=CARTESIAN_POINT('Ctrl Pts',(19.4378084870364,-21.4147872530806,-16.7312429631383));
#53243=CARTESIAN_POINT('Ctrl Pts',(19.356261744668,-21.435221762373,-16.7354125290823));
#53244=CARTESIAN_POINT('Ctrl Pts',(19.271847919437,-21.4563747238033,-16.7397286918212));
#53245=CARTESIAN_POINT('Ctrl Pts',(19.1863843882472,-21.4732110218617,-16.7440448545601));
#53246=CARTESIAN_POINT('Ctrl Pts',(19.1003501078358,-21.4856510411832,-16.7483610172991));
#53247=CARTESIAN_POINT('Ctrl Pts',(19.0171183850596,-21.4976858281838,-16.7525365814907));
#53248=CARTESIAN_POINT('Ctrl Pts',(18.9333529997362,-21.5056063582133,-16.7567121456824));
#53249=CARTESIAN_POINT('Ctrl Pts',(18.8494917538631,-21.5093935275568,-16.7608877098741));
#53250=CARTESIAN_POINT('Ctrl Pts',(18.7613948758223,-21.5133719778208,-16.7652741718866));
#53251=CARTESIAN_POINT('Ctrl Pts',(18.6731927827732,-21.5127885456943,-16.7696606338992));
#53252=CARTESIAN_POINT('Ctrl Pts',(18.5853894488633,-21.5076828645375,-16.7740470959117));
#53253=CARTESIAN_POINT('Ctrl Pts',(18.4975861149534,-21.5025771833808,-16.7784335579242));
#53254=CARTESIAN_POINT('Ctrl Pts',(18.4101821085832,-21.4929493923299,-16.7828200199368));
#53255=CARTESIAN_POINT('Ctrl Pts',(18.3236691980734,-21.4789009939035,-16.7872064819493));
#53256=CARTESIAN_POINT('Ctrl Pts',(18.2411368748189,-21.4654989831133,-16.7913911163424));
#53257=CARTESIAN_POINT('Ctrl Pts',(18.1591082470633,-21.4480243381486,-16.7955757507354));
#53258=CARTESIAN_POINT('Ctrl Pts',(18.0780163119226,-21.4265273085938,-16.7997603851285));
#53259=CARTESIAN_POINT('Ctrl Pts',(17.9970398011144,-21.4050608773998,-16.8039390632124));
#53260=CARTESIAN_POINT('Ctrl Pts',(17.9169977755054,-21.3795835508677,-16.8081177412964));
#53261=CARTESIAN_POINT('Ctrl Pts',(17.8383151283769,-21.3501969499492,-16.8122964193803));
#53262=CARTESIAN_POINT('Ctrl Pts',(17.7582221513468,-21.3202836153289,-16.8165499972658));
#53263=CARTESIAN_POINT('Ctrl Pts',(17.6795382417637,-21.2863195576311,-16.8208035751512));
#53264=CARTESIAN_POINT('Ctrl Pts',(17.6026975961514,-21.248465734786,-16.8250571530366));
#53265=CARTESIAN_POINT('Ctrl Pts',(17.5273466563964,-21.2113457821624,-16.8292282670146));
#53266=CARTESIAN_POINT('Ctrl Pts',(17.4537685795459,-21.1704857525209,-16.8333993809925));
#53267=CARTESIAN_POINT('Ctrl Pts',(17.3823529481854,-21.126086071737,-16.8375704949705));
#53268=CARTESIAN_POINT('Ctrl Pts',(17.3109612810297,-21.0817012896948,-16.8417402092909));
#53269=CARTESIAN_POINT('Ctrl Pts',(17.2417310086115,-21.0337794581179,-16.8459099236112));
#53270=CARTESIAN_POINT('Ctrl Pts',(17.1750254175657,-20.9825659928512,-16.8500796379316));
#53271=CARTESIAN_POINT('Ctrl Pts',(17.1083222001911,-20.9313543499794,-16.8542492038757));
#53272=CARTESIAN_POINT('Ctrl Pts',(17.0441438499404,-20.8768515871274,-16.8584187698197));
#53273=CARTESIAN_POINT('Ctrl Pts',(16.9828219564691,-20.8193444941562,-16.8625883357638));
#53274=CARTESIAN_POINT('Ctrl Pts',(16.9193440608722,-20.7598155227389,-16.8669044985027));
#53275=CARTESIAN_POINT('Ctrl Pts',(16.858927610118,-20.6970673867186,-16.8712206612416));
#53276=CARTESIAN_POINT('Ctrl Pts',(16.8018987983269,-20.6314597186278,-16.8755368239805));
#53277=CARTESIAN_POINT('Ctrl Pts',(16.7467276940815,-20.5679892134243,-16.8797123881722));
#53278=CARTESIAN_POINT('Ctrl Pts',(16.6947271674384,-20.5018430132072,-16.8838879523639));
#53279=CARTESIAN_POINT('Ctrl Pts',(16.6461502555163,-20.4333788996942,-16.8880635165556));
#53280=CARTESIAN_POINT('Ctrl Pts',(16.5951198392536,-20.3614568265656,-16.8924499785681));
#53281=CARTESIAN_POINT('Ctrl Pts',(16.5478682932594,-20.2869770238506,-16.8968364405806));
#53282=CARTESIAN_POINT('Ctrl Pts',(16.5046350837971,-20.210384706838,-16.9012229025932));
#53283=CARTESIAN_POINT('Ctrl Pts',(16.4614018743349,-20.1337923898254,-16.9056093646057));
#53284=CARTESIAN_POINT('Ctrl Pts',(16.4221871920777,-20.0550881117615,-16.9099958266183));
#53285=CARTESIAN_POINT('Ctrl Pts',(16.3871718743353,-19.9747403133684,-16.9143822886308));
#53286=CARTESIAN_POINT('Ctrl Pts',(16.3503471043863,-19.8902404606612,-16.9189954255353));
#53287=CARTESIAN_POINT('Ctrl Pts',(16.3180481684136,-19.8036540013278,-16.9236085624399));
#53288=CARTESIAN_POINT('Ctrl Pts',(16.290492039707,-19.7154584782324,-16.9282216993444));
#53289=CARTESIAN_POINT('Ctrl Pts',(16.2630147812854,-19.6275153855894,-16.9328216326736));
#53290=CARTESIAN_POINT('Ctrl Pts',(16.2402533773008,-19.5379726851084,-16.9374215660028));
#53291=CARTESIAN_POINT('Ctrl Pts',(16.2223767943064,-19.4473270360289,-16.9420214993319));
#53292=CARTESIAN_POINT('Ctrl Pts',(16.2045882581333,-19.3571278403507,-16.9465987767929));
#53293=CARTESIAN_POINT('Ctrl Pts',(16.1916366671696,-19.2658368103364,-16.9511760542539));
#53294=CARTESIAN_POINT('Ctrl Pts',(16.1836406660146,-19.17396231111,-16.9557533317148));
#53295=CARTESIAN_POINT('Ctrl Pts',(16.1772607284146,-19.100656472263,-16.9594055003442));
#53296=CARTESIAN_POINT('Ctrl Pts',(16.1740347749072,-19.0269796000837,-16.9630576689735));
#53297=CARTESIAN_POINT('Ctrl Pts',(16.1740002797795,-18.9531968587196,-16.9667098376028));
#53298=CARTESIAN_POINT('Origin',(18.734,-18.952,1.76670989022851));
#53299=CARTESIAN_POINT('',(20.295887153474,-16.918834963786,-15.6501589836526));
#53300=CARTESIAN_POINT('',(20.293535888361,-16.9218650751948,-15.7166572089129));
#53301=CARTESIAN_POINT('',(20.293535888361,-16.9218650751948,1.76670989022851));
#53302=CARTESIAN_POINT('',(16.1740007055014,-18.9500994299064,-16.2332901098004));
#53303=CARTESIAN_POINT('Ctrl Pts',(20.293535888361,-16.9218650751948,-15.7166572089129));
#53304=CARTESIAN_POINT('Ctrl Pts',(20.3624598556926,-16.9748119997112,-15.7209678975543));
#53305=CARTESIAN_POINT('Ctrl Pts',(20.428659775607,-17.0312538804154,-15.7252785861958));
#53306=CARTESIAN_POINT('Ctrl Pts',(20.4917771265502,-17.090866051737,-15.7295892748372));
#53307=CARTESIAN_POINT('Ctrl Pts',(20.5529161182364,-17.148609730652,-15.7337648486385));
#53308=CARTESIAN_POINT('Ctrl Pts',(20.6111626415143,-17.2093275174942,-15.7379404224398));
#53309=CARTESIAN_POINT('Ctrl Pts',(20.6662297662403,-17.2726881973693,-15.7421159962412));
#53310=CARTESIAN_POINT('Ctrl Pts',(20.7239697161052,-17.3391242515049,-15.7464942423026));
#53311=CARTESIAN_POINT('Ctrl Pts',(20.7782134511509,-17.4084658019913,-15.750872488364));
#53312=CARTESIAN_POINT('Ctrl Pts',(20.8286804992412,-17.4802956797988,-15.7552507344255));
#53313=CARTESIAN_POINT('Ctrl Pts',(20.8791475473314,-17.5521255576064,-15.7596289804869));
#53314=CARTESIAN_POINT('Ctrl Pts',(20.9258376665922,-17.626443235887,-15.7640072265483));
#53315=CARTESIAN_POINT('Ctrl Pts',(20.9685260259021,-17.7028028820213,-15.7683854726098));
#53316=CARTESIAN_POINT('Ctrl Pts',(21.0093266510939,-17.775785806455,-15.7725701070028));
#53317=CARTESIAN_POINT('Ctrl Pts',(21.0466238491571,-17.850905564207,-15.7767547413958));
#53318=CARTESIAN_POINT('Ctrl Pts',(21.0801878476017,-17.9277917283258,-15.7809393757889));
#53319=CARTESIAN_POINT('Ctrl Pts',(21.1137040718491,-18.0045684545067,-15.7851180538728));
#53320=CARTESIAN_POINT('Ctrl Pts',(21.1434974687763,-18.0831061749367,-15.7892967319568));
#53321=CARTESIAN_POINT('Ctrl Pts',(21.1693835453414,-18.1630088802273,-15.7934754100407));
#53322=CARTESIAN_POINT('Ctrl Pts',(21.195733611225,-18.2443437840852,-15.7977289879261));
#53323=CARTESIAN_POINT('Ctrl Pts',(21.218034666248,-18.3270926679896,-15.8019825658116));
#53324=CARTESIAN_POINT('Ctrl Pts',(21.2361429171342,-18.4108153529199,-15.806236143697));
#53325=CARTESIAN_POINT('Ctrl Pts',(21.2539001042416,-18.4929149102315,-15.810407257675));
#53326=CARTESIAN_POINT('Ctrl Pts',(21.2676255061034,-18.575950377106,-15.8145783716529));
#53327=CARTESIAN_POINT('Ctrl Pts',(21.2772339776254,-18.6594919914747,-15.8187494856309));
#53328=CARTESIAN_POINT('Ctrl Pts',(21.2868392249321,-18.7430055726479,-15.8229191999513));
#53329=CARTESIAN_POINT('Ctrl Pts',(21.2923302330118,-18.8270245073654,-15.8270889142716));
#53330=CARTESIAN_POINT('Ctrl Pts',(21.2936734448665,-18.9111116685929,-15.831258628592));
#53331=CARTESIAN_POINT('Ctrl Pts',(21.295016608924,-18.9951958376383,-15.8354281945361));
#53332=CARTESIAN_POINT('Ctrl Pts',(21.2922122637205,-19.0793477683788,-15.8395977604801));
#53333=CARTESIAN_POINT('Ctrl Pts',(21.285278964847,-19.1631294473285,-15.8437673264241));
#53334=CARTESIAN_POINT('Ctrl Pts',(21.2781018997383,-19.2498567867541,-15.8480834891631));
#53335=CARTESIAN_POINT('Ctrl Pts',(21.2665001742353,-19.3361868282291,-15.852399651902));
#53336=CARTESIAN_POINT('Ctrl Pts',(21.2505527597975,-19.421640508427,-15.8567158146409));
#53337=CARTESIAN_POINT('Ctrl Pts',(21.2351248307076,-19.5043105439806,-15.8608913788326));
#53338=CARTESIAN_POINT('Ctrl Pts',(21.2156301415435,-19.5861599891145,-15.8650669430243));
#53339=CARTESIAN_POINT('Ctrl Pts',(21.192191685782,-19.6667682393282,-15.8692425072159));
#53340=CARTESIAN_POINT('Ctrl Pts',(21.1675694093396,-19.7514478206323,-15.8736289692285));
#53341=CARTESIAN_POINT('Ctrl Pts',(21.1385946886759,-19.8347569748337,-15.878015431241));
#53342=CARTESIAN_POINT('Ctrl Pts',(21.1054674445918,-19.9162313826262,-15.8824018932535));
#53343=CARTESIAN_POINT('Ctrl Pts',(21.0723402005077,-19.9977057904187,-15.8867883552661));
#53344=CARTESIAN_POINT('Ctrl Pts',(21.0350607478796,-20.0773449585575,-15.8911748172786));
#53345=CARTESIAN_POINT('Ctrl Pts',(20.9938836431737,-20.1547160593073,-15.8955612792911));
#53346=CARTESIAN_POINT('Ctrl Pts',(20.9546011580944,-20.2285272010203,-15.8997459136842));
#53347=CARTESIAN_POINT('Ctrl Pts',(20.9116255956986,-20.3005491422943,-15.9039305480772));
#53348=CARTESIAN_POINT('Ctrl Pts',(20.8651440549404,-20.3703881757446,-15.9081151824703));
#53349=CARTESIAN_POINT('Ctrl Pts',(20.8187286749022,-20.4401278019752,-15.9122938605542));
#53350=CARTESIAN_POINT('Ctrl Pts',(20.7688174815646,-20.5076903123668,-15.9164725386382));
#53351=CARTESIAN_POINT('Ctrl Pts',(20.7156435935688,-20.5727062250969,-15.9206512167221));
#53352=CARTESIAN_POINT('Ctrl Pts',(20.6615166018461,-20.6388875013365,-15.9249047946076));
#53353=CARTESIAN_POINT('Ctrl Pts',(20.6040090238882,-20.7024295607932,-15.929158372493));
#53354=CARTESIAN_POINT('Ctrl Pts',(20.5434131480185,-20.7629732355222,-15.9334119503784));
#53355=CARTESIAN_POINT('Ctrl Pts',(20.4839920414457,-20.8223431529752,-15.9375830643564));
#53356=CARTESIAN_POINT('Ctrl Pts',(20.4216016541568,-20.878829567176,-15.9417541783343));
#53357=CARTESIAN_POINT('Ctrl Pts',(20.3565572606157,-20.9321282625181,-15.9459252923123));
#53358=CARTESIAN_POINT('Ctrl Pts',(20.2915346933491,-20.9854090729684,-15.9500950066327));
#53359=CARTESIAN_POINT('Ctrl Pts',(20.2238602440649,-21.0355039976099,-15.954264720953));
#53360=CARTESIAN_POINT('Ctrl Pts',(20.1538833036554,-21.0821482117451,-15.9584344352734));
#53361=CARTESIAN_POINT('Ctrl Pts',(20.0839088533259,-21.1287907660788,-15.9626040012174));
#53362=CARTESIAN_POINT('Ctrl Pts',(20.0116324580351,-21.1719825996021,-15.9667735671615));
#53363=CARTESIAN_POINT('Ctrl Pts',(19.937432461597,-21.211502226238,-15.9709431331055));
#53364=CARTESIAN_POINT('Ctrl Pts',(19.8606236848194,-21.2524113141939,-15.9752592958444));
#53365=CARTESIAN_POINT('Ctrl Pts',(19.7817539879933,-21.2893849131306,-15.9795754585833));
#53366=CARTESIAN_POINT('Ctrl Pts',(19.7012689333162,-21.3222301176555,-15.9838916213223));
#53367=CARTESIAN_POINT('Ctrl Pts',(19.6234056708299,-21.3540053930976,-15.9880671855139));
#53368=CARTESIAN_POINT('Ctrl Pts',(19.5440311349293,-21.3819169968656,-15.9922427497056));
#53369=CARTESIAN_POINT('Ctrl Pts',(19.4635655614735,-21.4058406817705,-15.9964183138973));
#53370=CARTESIAN_POINT('Ctrl Pts',(19.3790358631909,-21.4309726951269,-16.0008047759098));
#53371=CARTESIAN_POINT('Ctrl Pts',(19.2933025817205,-21.4517032054839,-16.0051912379224));
#53372=CARTESIAN_POINT('Ctrl Pts',(19.2068643494563,-21.4679489873631,-16.0095776999349));
#53373=CARTESIAN_POINT('Ctrl Pts',(19.1204261171922,-21.4841947692422,-16.0139641619475));
#53374=CARTESIAN_POINT('Ctrl Pts',(19.0332835193119,-21.4959558204205,-16.01835062396));
#53375=CARTESIAN_POINT('Ctrl Pts',(18.9459382820314,-21.5032119011579,-16.0227370859726));
#53376=CARTESIAN_POINT('Ctrl Pts',(18.862611928595,-21.5101341188644,-16.0269217203656));
#53377=CARTESIAN_POINT('Ctrl Pts',(18.7787910168741,-21.5129825827272,-16.0311063547587));
#53378=CARTESIAN_POINT('Ctrl Pts',(18.6949078655888,-21.5117015070174,-16.0352909891517));
#53379=CARTESIAN_POINT('Ctrl Pts',(18.6111441115866,-21.5104222547603,-16.0394696672357));
#53380=CARTESIAN_POINT('Ctrl Pts',(18.5273187500332,-21.5050251452316,-16.0436483453196));
#53381=CARTESIAN_POINT('Ctrl Pts',(18.4438686393689,-21.4955062008138,-16.0478270234036));
#53382=CARTESIAN_POINT('Ctrl Pts',(18.3589227454455,-21.4858166361585,-16.052080601289));
#53383=CARTESIAN_POINT('Ctrl Pts',(18.2743661679602,-21.4718559754809,-16.0563341791745));
#53384=CARTESIAN_POINT('Ctrl Pts',(18.1906591204409,-21.4536755762089,-16.0605877570599));
#53385=CARTESIAN_POINT('Ctrl Pts',(18.1085748973785,-21.4358476394529,-16.0647588710379));
#53386=CARTESIAN_POINT('Ctrl Pts',(18.0273080288923,-21.413962221893,-16.0689299850158));
#53387=CARTESIAN_POINT('Ctrl Pts',(17.9472849642516,-21.3881197533223,-16.0731010989937));
#53388=CARTESIAN_POINT('Ctrl Pts',(17.8672887521231,-21.3622859564417,-16.0772708133141));
#53389=CARTESIAN_POINT('Ctrl Pts',(17.7885359523432,-21.3324978868904,-16.0814405276345));
#53390=CARTESIAN_POINT('Ctrl Pts',(17.7114383592364,-21.2989059825308,-16.0856102419549));
#53391=CARTESIAN_POINT('Ctrl Pts',(17.634343509593,-21.2653152735153,-16.0897798078989));
#53392=CARTESIAN_POINT('Ctrl Pts',(17.558904170915,-21.2279211833515,-16.0939493738429));
#53393=CARTESIAN_POINT('Ctrl Pts',(17.485511368273,-21.1869219531,-16.098118939787));
#53394=CARTESIAN_POINT('Ctrl Pts',(17.4095381652297,-21.1444812404909,-16.1024351025259));
#53395=CARTESIAN_POINT('Ctrl Pts',(17.3357585487131,-21.098177414705,-16.1067512652648));
#53396=CARTESIAN_POINT('Ctrl Pts',(17.2645758959971,-21.0482807070083,-16.1110674280037));
#53397=CARTESIAN_POINT('Ctrl Pts',(17.1957120107063,-21.0000093793167,-16.1152429921954));
#53398=CARTESIAN_POINT('Ctrl Pts',(17.1292788382186,-20.948375977651,-16.1194185563871));
#53399=CARTESIAN_POINT('Ctrl Pts',(17.0656083164573,-20.8936666012181,-16.1235941205788));
#53400=CARTESIAN_POINT('Ctrl Pts',(16.9987219480043,-20.8361939842407,-16.1279805825913));
#53401=CARTESIAN_POINT('Ctrl Pts',(16.9348850702689,-20.7753268941812,-16.1323670446039));
#53402=CARTESIAN_POINT('Ctrl Pts',(16.8744375629656,-20.7114395535996,-16.1367535066164));
#53403=CARTESIAN_POINT('Ctrl Pts',(16.8139900556624,-20.647552213018,-16.141139968629));
#53404=CARTESIAN_POINT('Ctrl Pts',(16.7569322374057,-20.5806451127529,-16.1455264306415));
#53405=CARTESIAN_POINT('Ctrl Pts',(16.703552701499,-20.5111291697643,-16.149912892654));
#53406=CARTESIAN_POINT('Ctrl Pts',(16.6525544398241,-20.4447143500982,-16.1541036735168));
#53407=CARTESIAN_POINT('Ctrl Pts',(16.6047208600206,-20.3756679864259,-16.1582944543796));
#53408=CARTESIAN_POINT('Ctrl Pts',(16.5603345705066,-20.304323408296,-16.1624852352424));
#53409=CARTESIAN_POINT('Ctrl Pts',(16.516010837252,-20.2330793803581,-16.1666701097864));
#53410=CARTESIAN_POINT('Ctrl Pts',(16.4751249866854,-20.1595439541278,-16.1708549843304));
#53411=CARTESIAN_POINT('Ctrl Pts',(16.437918752824,-20.0840825528056,-16.1750398588744));
#53412=CARTESIAN_POINT('Ctrl Pts',(16.4007539244065,-20.0087051296905,-16.1792200762261));
#53413=CARTESIAN_POINT('Ctrl Pts',(16.3672607802463,-19.9314063968238,-16.1834002935778));
#53414=CARTESIAN_POINT('Ctrl Pts',(16.3376364602565,-19.8525785836828,-16.1875805109294));
#53415=CARTESIAN_POINT('Ctrl Pts',(16.3080359860442,-19.7738142221415,-16.1917573634601));
#53416=CARTESIAN_POINT('Ctrl Pts',(16.2822983085876,-19.6935236530688,-16.1959342159908));
#53417=CARTESIAN_POINT('Ctrl Pts',(16.2605729619717,-19.6121202068944,-16.2001110685215));
#53418=CARTESIAN_POINT('Ctrl Pts',(16.2388581016535,-19.5307560521889,-16.2042859049868));
#53419=CARTESIAN_POINT('Ctrl Pts',(16.2211518401956,-19.4482805298204,-16.2084607414521));
#53420=CARTESIAN_POINT('Ctrl Pts',(16.2075538451849,-19.3651220483341,-16.2126355779174));
#53421=CARTESIAN_POINT('Ctrl Pts',(16.1939550163507,-19.2819584676039,-16.216810670382));
#53422=CARTESIAN_POINT('Ctrl Pts',(16.1844650395067,-19.1981122945307,-16.2209857628465));
#53423=CARTESIAN_POINT('Ctrl Pts',(16.1791322578279,-19.1140210480408,-16.2251608553111));
#53424=CARTESIAN_POINT('Ctrl Pts',(16.1756711337436,-19.0594434830796,-16.2278706067979));
#53425=CARTESIAN_POINT('Ctrl Pts',(16.1739601228212,-19.0047628516759,-16.2305803582847));
#53426=CARTESIAN_POINT('Ctrl Pts',(16.174000705501,-18.9500994304892,-16.2332901097715));
#53427=CARTESIAN_POINT('Ctrl Pts',(16.1740007055014,-18.9500994299065,-16.2332901098004));
#53428=CARTESIAN_POINT('Ctrl Pts',(16.1740727513108,-18.8530563258851,-16.2381006886061));
#53429=CARTESIAN_POINT('Ctrl Pts',(16.1796667621363,-18.7562381388328,-16.2429112674118));
#53430=CARTESIAN_POINT('Ctrl Pts',(16.1906824963738,-18.6602191305988,-16.2477218462176));
#53431=CARTESIAN_POINT('Ctrl Pts',(16.2018903455192,-18.5625255464786,-16.2526163217372));
#53432=CARTESIAN_POINT('Ctrl Pts',(16.2187106399962,-18.465659449398,-16.2575107972569));
#53433=CARTESIAN_POINT('Ctrl Pts',(16.2409867483463,-18.3702054253614,-16.2624052727765));
#53434=CARTESIAN_POINT('Ctrl Pts',(16.2632628566963,-18.2747514013248,-16.2672997482962));
#53435=CARTESIAN_POINT('Ctrl Pts',(16.2909946214078,-18.1807095711099,-16.2721942238158));
#53436=CARTESIAN_POINT('Ctrl Pts',(16.3239764935689,-18.088642195582,-16.2770886993355));
#53437=CARTESIAN_POINT('Ctrl Pts',(16.3521750361989,-18.0099272639074,-16.2812733337285));
#53438=CARTESIAN_POINT('Ctrl Pts',(16.3842865295797,-17.9324488089606,-16.2854579681216));
#53439=CARTESIAN_POINT('Ctrl Pts',(16.4201827606336,-17.8566234515881,-16.2896426025146));
#53440=CARTESIAN_POINT('Ctrl Pts',(16.4560278978456,-17.7809060222267,-16.2938212805986));
#53441=CARTESIAN_POINT('Ctrl Pts',(16.4956468770877,-17.7068374289188,-16.2979999586825));
#53442=CARTESIAN_POINT('Ctrl Pts',(16.5388624466768,-17.6348169747563,-16.3021786367664));
#53443=CARTESIAN_POINT('Ctrl Pts',(16.5828526242923,-17.561505605713,-16.3064322146519));
#53444=CARTESIAN_POINT('Ctrl Pts',(16.6305694356435,-17.4903169777092,-16.3106857925373));
#53445=CARTESIAN_POINT('Ctrl Pts',(16.6817755898823,-17.4216487427662,-16.3149393704227));
#53446=CARTESIAN_POINT('Ctrl Pts',(16.7319890129005,-17.3543117755527,-16.3191104844007));
#53447=CARTESIAN_POINT('Ctrl Pts',(16.7855574030481,-17.289398733779,-16.3232815983786));
#53448=CARTESIAN_POINT('Ctrl Pts',(16.8422127801053,-17.2272562176824,-16.3274527123566));
#53449=CARTESIAN_POINT('Ctrl Pts',(16.8988491459036,-17.1651345541072,-16.331622426677));
#53450=CARTESIAN_POINT('Ctrl Pts',(16.9585701316816,-17.1057819095285,-16.3357921409973));
#53451=CARTESIAN_POINT('Ctrl Pts',(17.0210683042877,-17.0495108394989,-16.3399618553177));
#53452=CARTESIAN_POINT('Ctrl Pts',(17.0835642529406,-16.9932417718355,-16.3441314212617));
#53453=CARTESIAN_POINT('Ctrl Pts',(17.1488368494855,-16.9400543678788,-16.3483009872058));
#53454=CARTESIAN_POINT('Ctrl Pts',(17.2165437463576,-16.8902224857465,-16.3524705531498));
#53455=CARTESIAN_POINT('Ctrl Pts',(17.2866311341982,-16.8386385761127,-16.3567867158888));
#53456=CARTESIAN_POINT('Ctrl Pts',(17.3593267625534,-16.790650851497,-16.3611028786277));
#53457=CARTESIAN_POINT('Ctrl Pts',(17.4342176396319,-16.7465146076938,-16.3654190413666));
#53458=CARTESIAN_POINT('Ctrl Pts',(17.5066689542667,-16.7038160973902,-16.3695946055583));
#53459=CARTESIAN_POINT('Ctrl Pts',(17.5811742544606,-16.664722174367,-16.37377016975));
#53460=CARTESIAN_POINT('Ctrl Pts',(17.6573356824289,-16.6294165359951,-16.3779457339416));
#53461=CARTESIAN_POINT('Ctrl Pts',(17.7373438430673,-16.5923276937602,-16.3823321959542));
#53462=CARTESIAN_POINT('Ctrl Pts',(17.8191792885611,-16.5594201038736,-16.3867186579667));
#53463=CARTESIAN_POINT('Ctrl Pts',(17.902360657527,-16.5308482071437,-16.3911051199793));
#53464=CARTESIAN_POINT('Ctrl Pts',(17.985542026493,-16.5022763104139,-16.3954915819918));
#53465=CARTESIAN_POINT('Ctrl Pts',(18.0700687402227,-16.4780401936422,-16.3998780440043));
#53466=CARTESIAN_POINT('Ctrl Pts',(18.155447269861,-16.4582324209244,-16.4042645060169));
#53467=CARTESIAN_POINT('Ctrl Pts',(18.2369040239202,-16.4393344980206,-16.4084494803759));
#53468=CARTESIAN_POINT('Ctrl Pts',(18.3194392781939,-16.4243966729015,-16.4126344547349));
#53469=CARTESIAN_POINT('Ctrl Pts',(18.4026332182035,-16.4135366743004,-16.4168194290939));
#53470=CARTESIAN_POINT('Ctrl Pts',(18.4856850454026,-16.4026952268693,-16.4209972546333));
#53471=CARTESIAN_POINT('Ctrl Pts',(18.5693928687512,-16.3959178140199,-16.4251750801727));
#53472=CARTESIAN_POINT('Ctrl Pts',(18.6533252588854,-16.3932714903402,-16.4293529057121));
#53473=CARTESIAN_POINT('Ctrl Pts',(18.7371760689814,-16.3906277388162,-16.4335266705169));
#53474=CARTESIAN_POINT('Ctrl Pts',(18.821250555471,-16.3921071193265,-16.4377004353216));
#53475=CARTESIAN_POINT('Ctrl Pts',(18.9051115090561,-16.3977249851536,-16.4418742001264));
#53476=CARTESIAN_POINT('Ctrl Pts',(18.9889161108074,-16.4033390759575,-16.4460451602969));
#53477=CARTESIAN_POINT('Ctrl Pts',(19.0725070069923,-16.4130860985607,-16.4502161204674));
#53478=CARTESIAN_POINT('Ctrl Pts',(19.1554476929898,-16.426929339192,-16.4543870806379));
#53479=CARTESIAN_POINT('Ctrl Pts',(19.238357526517,-16.4407674303823,-16.4585564892849));
#53480=CARTESIAN_POINT('Ctrl Pts',(19.3206171772897,-16.4586986359201,-16.4627258979319));
#53481=CARTESIAN_POINT('Ctrl Pts',(19.4017973253963,-16.480634642107,-16.4668953065789));
#53482=CARTESIAN_POINT('Ctrl Pts',(19.4830102717198,-16.5025795108288,-16.4710663997408));
#53483=CARTESIAN_POINT('Ctrl Pts',(19.5631423969829,-16.5285323016481,-16.4752374929027));
#53484=CARTESIAN_POINT('Ctrl Pts',(19.6417773433661,-16.5583541834952,-16.4794085860646));
#53485=CARTESIAN_POINT('Ctrl Pts',(19.7204244341719,-16.5881806710494,-16.4835803234123));
#53486=CARTESIAN_POINT('Ctrl Pts',(19.7975734594219,-16.6218772648632,-16.48775206076));
#53487=CARTESIAN_POINT('Ctrl Pts',(19.8728278889775,-16.6592568745524,-16.4919237981077));
#53488=CARTESIAN_POINT('Ctrl Pts',(19.9481771492369,-16.6966835875779,-16.4961007924057));
#53489=CARTESIAN_POINT('Ctrl Pts',(20.0216266360836,-16.7378023734385,-16.5002777867036));
#53490=CARTESIAN_POINT('Ctrl Pts',(20.0928045893757,-16.7823801973867,-16.5044547810015));
#53491=CARTESIAN_POINT('Ctrl Pts',(20.1619637771322,-16.8256936948059,-16.5085133064234));
#53492=CARTESIAN_POINT('Ctrl Pts',(20.2289782742483,-16.8722723536246,-16.5125718318452));
#53493=CARTESIAN_POINT('Ctrl Pts',(20.293535888361,-16.9218650751947,-16.516630357267));
#53494=CARTESIAN_POINT('',(16.1740005630998,-18.9536979607663,-16.1667098902285));
#53495=CARTESIAN_POINT('Ctrl Pts',(16.1740005630998,-18.9536979607663,-16.1667098902285));
#53496=CARTESIAN_POINT('Ctrl Pts',(16.1739457994085,-18.8711312597184,-16.1708335669039));
#53497=CARTESIAN_POINT('Ctrl Pts',(16.1778897355288,-18.7884072256501,-16.1749572435793));
#53498=CARTESIAN_POINT('Ctrl Pts',(16.185851592152,-18.7059518510905,-16.1790809202548));
#53499=CARTESIAN_POINT('Ctrl Pts',(16.193849980064,-18.6231181475504,-16.1832235175451));
#53500=CARTESIAN_POINT('Ctrl Pts',(16.2059033176551,-18.5405560554534,-16.1873661148355));
#53501=CARTESIAN_POINT('Ctrl Pts',(16.2219780566694,-18.4586991220099,-16.1915087121259));
#53502=CARTESIAN_POINT('Ctrl Pts',(16.23794569149,-18.3773875921872,-16.1956237077524));
#53503=CARTESIAN_POINT('Ctrl Pts',(16.2578812222445,-18.2967723256482,-16.1997387033789));
#53504=CARTESIAN_POINT('Ctrl Pts',(16.2816998746989,-18.2172727748012,-16.2038536990054));
#53505=CARTESIAN_POINT('Ctrl Pts',(16.3055083094402,-18.1378073276299,-16.2079669293832));
#53506=CARTESIAN_POINT('Ctrl Pts',(16.33319642467,-18.0594570997615,-16.2120801597611));
#53507=CARTESIAN_POINT('Ctrl Pts',(16.3646289972004,-17.9826285278118,-16.2161933901389));
#53508=CARTESIAN_POINT('Ctrl Pts',(16.3960581246075,-17.9058083765508,-16.2203061696919));
#53509=CARTESIAN_POINT('Ctrl Pts',(16.4312307139714,-17.8305099882011,-16.2244189492448));
#53510=CARTESIAN_POINT('Ctrl Pts',(16.4699631644818,-17.7571204213743,-16.2285317287977));
#53511=CARTESIAN_POINT('Ctrl Pts',(16.5091807554343,-17.6828116189603,-16.2326960226666));
#53512=CARTESIAN_POINT('Ctrl Pts',(16.5520477937181,-17.6104602387452,-16.2368603165354));
#53513=CARTESIAN_POINT('Ctrl Pts',(16.5983263505015,-17.5404412648289,-16.2410246104042));
#53514=CARTESIAN_POINT('Ctrl Pts',(16.6440925485816,-17.4711974842891,-16.2451428005836));
#53515=CARTESIAN_POINT('Ctrl Pts',(16.6931947649454,-17.404235069768,-16.2492609907631));
#53516=CARTESIAN_POINT('Ctrl Pts',(16.7453611252722,-17.3398847975652,-16.2533791809425));
#53517=CARTESIAN_POINT('Ctrl Pts',(16.7984034996616,-17.2744539105174,-16.257566526656));
#53518=CARTESIAN_POINT('Ctrl Pts',(16.8546135316781,-17.2117240820489,-16.2617538723695));
#53519=CARTESIAN_POINT('Ctrl Pts',(16.9136665630955,-17.1520038393131,-16.265941218083));
#53520=CARTESIAN_POINT('Ctrl Pts',(16.9727195945129,-17.0922835965773,-16.2701285637965));
#53521=CARTESIAN_POINT('Ctrl Pts',(17.0346152026565,-17.0355732283015,-16.27431590951));
#53522=CARTESIAN_POINT('Ctrl Pts',(17.098995528925,-16.9821369642626,-16.2785032552236));
#53523=CARTESIAN_POINT('Ctrl Pts',(17.1633341687151,-16.9287353003848,-16.2826878896166));
#53524=CARTESIAN_POINT('Ctrl Pts',(17.2304115572044,-16.8783896656035,-16.2868725240096));
#53525=CARTESIAN_POINT('Ctrl Pts',(17.2999052707799,-16.8313934104547,-16.2910571584027));
#53526=CARTESIAN_POINT('Ctrl Pts',(17.3693000686557,-16.7844640486581,-16.2952358364866));
#53527=CARTESIAN_POINT('Ctrl Pts',(17.4411039821924,-16.7408748523863,-16.2994145145706));
#53528=CARTESIAN_POINT('Ctrl Pts',(17.5149611920067,-16.7008793047448,-16.3035931926545));
#53529=CARTESIAN_POINT('Ctrl Pts',(17.5901422392268,-16.6601668656561,-16.3078467705399));
#53530=CARTESIAN_POINT('Ctrl Pts',(17.6674505464318,-16.6231784826193,-16.3121003484254));
#53531=CARTESIAN_POINT('Ctrl Pts',(17.746479455157,-16.5901356572587,-16.3163539263108));
#53532=CARTESIAN_POINT('Ctrl Pts',(17.8239762342743,-16.5577334315455,-16.3205250402888));
#53533=CARTESIAN_POINT('Ctrl Pts',(17.9031270518497,-16.5291253296779,-16.3246961542667));
#53534=CARTESIAN_POINT('Ctrl Pts',(17.9835248188147,-16.5044732887209,-16.3288672682447));
#53535=CARTESIAN_POINT('Ctrl Pts',(18.0638956075326,-16.4798295199942,-16.333036982565));
#53536=CARTESIAN_POINT('Ctrl Pts',(18.1455120751843,-16.4591393105014,-16.3372066968854));
#53537=CARTESIAN_POINT('Ctrl Pts',(18.2279505020326,-16.4425152111226,-16.3413764112058));
#53538=CARTESIAN_POINT('Ctrl Pts',(18.3103859953678,-16.4258917033007,-16.3455459771498));
#53539=CARTESIAN_POINT('Ctrl Pts',(18.3936429386218,-16.4133341080144,-16.3497155430939));
#53540=CARTESIAN_POINT('Ctrl Pts',(18.4772872562555,-16.404903895178,-16.3538851090379));
#53541=CARTESIAN_POINT('Ctrl Pts',(18.563872404911,-16.3961772864581,-16.3582012717768));
#53542=CARTESIAN_POINT('Ctrl Pts',(18.6508721501762,-16.3918737507556,-16.3625174345158));
#53543=CARTESIAN_POINT('Ctrl Pts',(18.7378010569178,-16.3920028218831,-16.3668335972547));
#53544=CARTESIAN_POINT('Ctrl Pts',(18.8218982636656,-16.3921276885323,-16.3710091614464));
#53545=CARTESIAN_POINT('Ctrl Pts',(18.9059287081098,-16.3964007414036,-16.3751847256381));
#53546=CARTESIAN_POINT('Ctrl Pts',(18.9894564259426,-16.4047775883436,-16.3793602898297));
#53547=CARTESIAN_POINT('Ctrl Pts',(19.077202930235,-16.4135775299085,-16.3837467518423));
#53548=CARTESIAN_POINT('Ctrl Pts',(19.1643940106306,-16.4269066375599,-16.3881332138548));
#53549=CARTESIAN_POINT('Ctrl Pts',(19.2505367177893,-16.4446528323394,-16.3925196758674));
#53550=CARTESIAN_POINT('Ctrl Pts',(19.336679424948,-16.462399027119,-16.3969061378799));
#53551=CARTESIAN_POINT('Ctrl Pts',(19.4217732165569,-16.4845620891763,-16.4012925998925));
#53552=CARTESIAN_POINT('Ctrl Pts',(19.5053461655912,-16.510970485056,-16.405679061905));
#53553=CARTESIAN_POINT('Ctrl Pts',(19.5850559562966,-16.5361581532281,-16.4098627597761));
#53554=CARTESIAN_POINT('Ctrl Pts',(19.6636790298742,-16.5653010733602,-16.4140464576472));
#53555=CARTESIAN_POINT('Ctrl Pts',(19.7407944846487,-16.5982870043948,-16.4182301555183));
#53556=CARTESIAN_POINT('Ctrl Pts',(19.817813812666,-16.6312318174641,-16.4224086382829));
#53557=CARTESIAN_POINT('Ctrl Pts',(19.8933288322728,-16.668009955813,-16.4265871210475));
#53558=CARTESIAN_POINT('Ctrl Pts',(19.9669338586819,-16.7084594721477,-16.4307656038121));
#53559=CARTESIAN_POINT('Ctrl Pts',(20.0404561874598,-16.7488635421407,-16.434939391916));
#53560=CARTESIAN_POINT('Ctrl Pts',(20.1120723866515,-16.7929305724585,-16.4391131800199));
#53561=CARTESIAN_POINT('Ctrl Pts',(20.1813982979639,-16.8404512397174,-16.4432869681238));
#53562=CARTESIAN_POINT('Ctrl Pts',(20.2194886451346,-16.8665609392425,-16.4455802093504));
#53563=CARTESIAN_POINT('Ctrl Pts',(20.2568879854969,-16.8937124046252,-16.447873450577));
#53564=CARTESIAN_POINT('Ctrl Pts',(20.293535888361,-16.9218650751947,-16.4501666918036));
#53565=CARTESIAN_POINT('Ctrl Pts',(20.295887153474,-16.918834963786,-15.6501589836526));
#53566=CARTESIAN_POINT('Ctrl Pts',(20.9266956757797,-17.4084201070463,-15.6900393319344));
#53567=CARTESIAN_POINT('Ctrl Pts',(21.731566631022,-19.0750468017155,-15.7723116157766));
#53568=CARTESIAN_POINT('Ctrl Pts',(20.3102572374462,-21.5363190520979,-15.8969758351793));
#53569=CARTESIAN_POINT('Ctrl Pts',(17.414194801089,-21.6762257759895,-16.0241516418607));
#53570=CARTESIAN_POINT('Ctrl Pts',(16.2227678370508,-20.0081650868305,-16.1140629935438));
#53571=CARTESIAN_POINT('Ctrl Pts',(16.1704459057083,-19.0564768309817,-16.1615824096664));
#53572=CARTESIAN_POINT('Ctrl Pts',(16.1712325076282,-18.9536997967236,-16.1667098902285));
#53573=CARTESIAN_POINT('Origin',(18.734,-18.952,1.76670989022851));
#53574=CARTESIAN_POINT('',(20.2935358883611,-16.9218650751948,-14.8500370296196));
#53575=CARTESIAN_POINT('',(20.293535888361,-16.9218650751948,-14.9167585823994));
#53576=CARTESIAN_POINT('',(20.293535888361,-16.9218650751948,1.76670989022851));
#53577=CARTESIAN_POINT('',(16.174000571626,-18.9537107672549,-15.4332901097416));
#53578=CARTESIAN_POINT('Ctrl Pts',(20.293535888361,-16.9218650751948,-14.9167585823994));
#53579=CARTESIAN_POINT('Ctrl Pts',(20.3601520173691,-16.9730391339543,-14.92092957676));
#53580=CARTESIAN_POINT('Ctrl Pts',(20.4242947459017,-17.0275324319862,-14.9251005711207));
#53581=CARTESIAN_POINT('Ctrl Pts',(20.4856216570591,-17.0850716214805,-14.9292715654813));
#53582=CARTESIAN_POINT('Ctrl Pts',(20.5469290962655,-17.1425925416659,-14.9334412355066));
#53583=CARTESIAN_POINT('Ctrl Pts',(20.6054221585251,-17.2031571180328,-14.9376109055319));
#53584=CARTESIAN_POINT('Ctrl Pts',(20.6607930947023,-17.2664530946285,-14.9417805755571));
#53585=CARTESIAN_POINT('Ctrl Pts',(20.7161630599139,-17.3297479612879,-14.9459501724645));
#53586=CARTESIAN_POINT('Ctrl Pts',(20.7684107058034,-17.395773785992,-14.9501197693719));
#53587=CARTESIAN_POINT('Ctrl Pts',(20.8172675301325,-17.4641840174619,-14.9542893662793));
#53588=CARTESIAN_POINT('Ctrl Pts',(20.8671067638701,-17.5339698368045,-14.9585428051328));
#53589=CARTESIAN_POINT('Ctrl Pts',(20.9134170197272,-17.6062366054209,-14.9627962439863));
#53590=CARTESIAN_POINT('Ctrl Pts',(20.9559598088395,-17.6805855876616,-14.9670496828397));
#53591=CARTESIAN_POINT('Ctrl Pts',(20.9977248092744,-17.7535752843976,-14.9712253581838));
#53592=CARTESIAN_POINT('Ctrl Pts',(21.0358587906801,-17.8285712512628,-14.9754010335279));
#53593=CARTESIAN_POINT('Ctrl Pts',(21.0701835580393,-17.905173183785,-14.979576708872));
#53594=CARTESIAN_POINT('Ctrl Pts',(21.1054671694712,-17.9839149504446,-14.9838690294802));
#53595=CARTESIAN_POINT('Ctrl Pts',(21.1367253892166,-18.0643532541545,-14.9881613500884));
#53596=CARTESIAN_POINT('Ctrl Pts',(21.163819136657,-18.1460353834469,-14.9924536706966));
#53597=CARTESIAN_POINT('Ctrl Pts',(21.1909128840974,-18.2277175127393,-14.9967459913047));
#53598=CARTESIAN_POINT('Ctrl Pts',(21.213842087396,-18.3106429475775,-15.0010383119129));
#53599=CARTESIAN_POINT('Ctrl Pts',(21.2325245180281,-18.3943484665022,-15.0053306325211));
#53600=CARTESIAN_POINT('Ctrl Pts',(21.25073824177,-18.4759539720913,-15.0095152669141));
#53601=CARTESIAN_POINT('Ctrl Pts',(21.2649836214983,-18.5586046111965,-15.0136999013072));
#53602=CARTESIAN_POINT('Ctrl Pts',(21.2751464736302,-18.6418797014761,-15.0178845357002));
#53603=CARTESIAN_POINT('Ctrl Pts',(21.2852948602001,-18.725036259972,-15.0220632137842));
#53604=CARTESIAN_POINT('Ctrl Pts',(21.2913722063418,-18.8088150514091,-15.0262418918681));
#53605=CARTESIAN_POINT('Ctrl Pts',(21.2933150345072,-18.8927838354387,-15.0304205699521));
#53606=CARTESIAN_POINT('Ctrl Pts',(21.2952926864712,-18.9782576995749,-15.0346741478375));
#53607=CARTESIAN_POINT('Ctrl Pts',(21.2929860350544,-19.0639279639717,-15.0389277257229));
#53608=CARTESIAN_POINT('Ctrl Pts',(21.2863832385264,-19.1493317097919,-15.0431813036084));
#53609=CARTESIAN_POINT('Ctrl Pts',(21.2799084500935,-19.2330797373477,-15.0473524175863));
#53610=CARTESIAN_POINT('Ctrl Pts',(21.2693026454397,-19.3165710082865,-15.0515235315643));
#53611=CARTESIAN_POINT('Ctrl Pts',(21.2546071988876,-19.3993693651963,-15.0556946455422));
#53612=CARTESIAN_POINT('Ctrl Pts',(21.2399166835345,-19.4821399383178,-15.0598643598626));
#53613=CARTESIAN_POINT('Ctrl Pts',(21.2211393320557,-19.5642176066098,-15.064034074183));
#53614=CARTESIAN_POINT('Ctrl Pts',(21.1983680574964,-19.6451739155445,-15.0682037885034));
#53615=CARTESIAN_POINT('Ctrl Pts',(21.1755975932368,-19.7261273437063,-15.0723733544474));
#53616=CARTESIAN_POINT('Ctrl Pts',(21.1488336138537,-19.8059590492309,-15.0765429203915));
#53617=CARTESIAN_POINT('Ctrl Pts',(21.1182192201024,-19.8842546382263,-15.0807124863355));
#53618=CARTESIAN_POINT('Ctrl Pts',(21.0865284620338,-19.9653030035426,-15.0850286490744));
#53619=CARTESIAN_POINT('Ctrl Pts',(21.0507116827588,-20.0447047315976,-15.0893448118133));
#53620=CARTESIAN_POINT('Ctrl Pts',(21.0109816181364,-20.1220233803941,-15.0936609745523));
#53621=CARTESIAN_POINT('Ctrl Pts',(20.9725457561902,-20.1968233823388,-15.0978365387439));
#53622=CARTESIAN_POINT('Ctrl Pts',(20.9304479207722,-20.2696735493082,-15.1020121029356));
#53623=CARTESIAN_POINT('Ctrl Pts',(20.8849263037079,-20.3402060495537,-15.1061876671273));
#53624=CARTESIAN_POINT('Ctrl Pts',(20.8371054979832,-20.4143009787113,-15.1105741291398));
#53625=CARTESIAN_POINT('Ctrl Pts',(20.7855062921192,-20.4858374838363,-15.1149605911524));
#53626=CARTESIAN_POINT('Ctrl Pts',(20.7304530967375,-20.5544278556389,-15.1193470531649));
#53627=CARTESIAN_POINT('Ctrl Pts',(20.6753999013558,-20.6230182274415,-15.1237335151775));
#53628=CARTESIAN_POINT('Ctrl Pts',(20.6168931592929,-20.6886620833861,-15.12811997719));
#53629=CARTESIAN_POINT('Ctrl Pts',(20.5553006227462,-20.7510175211999,-15.1325064392025));
#53630=CARTESIAN_POINT('Ctrl Pts',(20.4965420501079,-20.810503892887,-15.1366910735956));
#53631=CARTESIAN_POINT('Ctrl Pts',(20.4347566962297,-20.8672192262126,-15.1408757079886));
#53632=CARTESIAN_POINT('Ctrl Pts',(20.3702364829786,-20.9208398034807,-15.1450603423817));
#53633=CARTESIAN_POINT('Ctrl Pts',(20.3058081062651,-20.9743840584939,-15.1492390204656));
#53634=CARTESIAN_POINT('Ctrl Pts',(20.2386529531481,-21.0248420156527,-15.1534176985496));
#53635=CARTESIAN_POINT('Ctrl Pts',(20.1691001101646,-21.0719263368819,-15.1575963766335));
#53636=CARTESIAN_POINT('Ctrl Pts',(20.0983005824574,-21.1198546107302,-15.1618499545189));
#53637=CARTESIAN_POINT('Ctrl Pts',(20.0250169010501,-21.1642867711771,-15.1661035324044));
#53638=CARTESIAN_POINT('Ctrl Pts',(19.9496318977225,-21.2049622920146,-15.1703571102898));
#53639=CARTESIAN_POINT('Ctrl Pts',(19.8757083797861,-21.2448492385089,-15.1745282242678));
#53640=CARTESIAN_POINT('Ctrl Pts',(19.7997647128025,-21.281123676622,-15.1786993382457));
#53641=CARTESIAN_POINT('Ctrl Pts',(19.722190031268,-21.3135843118768,-15.1828704522237));
#53642=CARTESIAN_POINT('Ctrl Pts',(19.6446413806671,-21.3460340546519,-15.1870401665441));
#53643=CARTESIAN_POINT('Ctrl Pts',(19.5654632264914,-21.3746723587588,-15.1912098808644));
#53644=CARTESIAN_POINT('Ctrl Pts',(19.4850661232634,-21.3993454350553,-15.1953795951848));
#53645=CARTESIAN_POINT('Ctrl Pts',(19.4046718809095,-21.4240176333779,-15.1995491611288));
#53646=CARTESIAN_POINT('Ctrl Pts',(19.3230592157836,-21.4447247502806,-15.2037187270729));
#53647=CARTESIAN_POINT('Ctrl Pts',(19.2406540252945,-21.4613628072985,-15.2078882930169));
#53648=CARTESIAN_POINT('Ctrl Pts',(19.1553515699655,-21.4785858378759,-15.2122044557559));
#53649=CARTESIAN_POINT('Ctrl Pts',(19.0692003389645,-21.4914482440571,-15.2165206184948));
#53650=CARTESIAN_POINT('Ctrl Pts',(18.9826824608282,-21.4998926652582,-15.2208367812337));
#53651=CARTESIAN_POINT('Ctrl Pts',(18.8989828934722,-21.5080620103268,-15.2250123454254));
#53652=CARTESIAN_POINT('Ctrl Pts',(18.8149406719769,-21.512096806535,-15.2291879096171));
#53653=CARTESIAN_POINT('Ctrl Pts',(18.7309940133496,-21.5119982351643,-15.2333634738087));
#53654=CARTESIAN_POINT('Ctrl Pts',(18.6428074085592,-21.5118946851879,-15.2377499358213));
#53655=CARTESIAN_POINT('Ctrl Pts',(18.5547268571684,-21.5072292722347,-15.2421363978338));
#53656=CARTESIAN_POINT('Ctrl Pts',(18.4672539586503,-21.4980649146132,-15.2465228598464));
#53657=CARTESIAN_POINT('Ctrl Pts',(18.3797810601321,-21.4889005569917,-15.2509093218589));
#53658=CARTESIAN_POINT('Ctrl Pts',(18.2929163758375,-21.4752374199981,-15.2552957838715));
#53659=CARTESIAN_POINT('Ctrl Pts',(18.20714644876,-21.4571996598167,-15.259682245884));
#53660=CARTESIAN_POINT('Ctrl Pts',(18.125322923169,-21.4399918437196,-15.263866880277));
#53661=CARTESIAN_POINT('Ctrl Pts',(18.0441910630359,-21.41873907309,-15.2680515146701));
#53662=CARTESIAN_POINT('Ctrl Pts',(17.9641810754837,-21.3935115857715,-15.2722361490631));
#53663=CARTESIAN_POINT('Ctrl Pts',(17.8842849722453,-21.3683200066586,-15.2764148271471));
#53664=CARTESIAN_POINT('Ctrl Pts',(17.8055080047354,-21.3391650856198,-15.280593505231));
#53665=CARTESIAN_POINT('Ctrl Pts',(17.728269907104,-21.3061680017032,-15.284772183315));
#53666=CARTESIAN_POINT('Ctrl Pts',(17.6496473720827,-21.2725794687721,-15.2890257612004));
#53667=CARTESIAN_POINT('Ctrl Pts',(17.5726198898779,-21.2350097758299,-15.2932793390859));
#53668=CARTESIAN_POINT('Ctrl Pts',(17.4976137413827,-21.1936398059239,-15.2975329169713));
#53669=CARTESIAN_POINT('Ctrl Pts',(17.4240617334387,-21.1530718736114,-15.3017040309492));
#53670=CARTESIAN_POINT('Ctrl Pts',(17.3524538049873,-21.1088499333756,-15.3058751449272));
#53671=CARTESIAN_POINT('Ctrl Pts',(17.2831698439507,-21.0611922288634,-15.3100462589051));
#53672=CARTESIAN_POINT('Ctrl Pts',(17.2139091318162,-21.0135505163542,-15.3142159732255));
#53673=CARTESIAN_POINT('Ctrl Pts',(17.1469712170494,-20.9624755897518,-15.3183856875459));
#53674=CARTESIAN_POINT('Ctrl Pts',(17.0827076373574,-20.9082294172919,-15.3225554018663));
#53675=CARTESIAN_POINT('Ctrl Pts',(17.0184463444393,-20.8539851751436,-15.3267249678103));
#53676=CARTESIAN_POINT('Ctrl Pts',(16.9568595483704,-20.7965702088949,-15.3308945337544));
#53677=CARTESIAN_POINT('Ctrl Pts',(16.8982652087742,-20.7362863492957,-15.3350640996984));
#53678=CARTESIAN_POINT('Ctrl Pts',(16.8376107644816,-20.6738829835612,-15.3393802624373));
#53679=CARTESIAN_POINT('Ctrl Pts',(16.7801634890496,-20.6084056085283,-15.3436964251763));
#53680=CARTESIAN_POINT('Ctrl Pts',(16.7262325806843,-20.5402285698017,-15.3480125879152));
#53681=CARTESIAN_POINT('Ctrl Pts',(16.6740584659864,-20.4742723909407,-15.3521881521069));
#53682=CARTESIAN_POINT('Ctrl Pts',(16.6251753803869,-20.4057901412944,-15.3563637162985));
#53683=CARTESIAN_POINT('Ctrl Pts',(16.5798195291698,-20.335150931422,-15.3605392804902));
#53684=CARTESIAN_POINT('Ctrl Pts',(16.532172861731,-20.2609439029878,-15.3649257425028));
#53685=CARTESIAN_POINT('Ctrl Pts',(16.488419403819,-20.1843567987727,-15.3693122045153));
#53686=CARTESIAN_POINT('Ctrl Pts',(16.4487777573746,-20.1058454410405,-15.3736986665278));
#53687=CARTESIAN_POINT('Ctrl Pts',(16.4091361109301,-20.0273340833083,-15.3780851285404));
#53688=CARTESIAN_POINT('Ctrl Pts',(16.3736064408137,-19.9468990335382,-15.3824715905529));
#53689=CARTESIAN_POINT('Ctrl Pts',(16.3423477078172,-19.8650166007783,-15.3868580525655));
#53690=CARTESIAN_POINT('Ctrl Pts',(16.3083133302778,-19.7758633510063,-15.3916340140292));
#53691=CARTESIAN_POINT('Ctrl Pts',(16.2792349760223,-19.6847190703936,-15.396409975493));
#53692=CARTESIAN_POINT('Ctrl Pts',(16.2553188691393,-19.5921092496716,-15.4011859369567));
#53693=CARTESIAN_POINT('Ctrl Pts',(16.2315006236314,-19.4998783754247,-15.405942355852));
#53694=CARTESIAN_POINT('Ctrl Pts',(16.212802591162,-19.406194112186,-15.4106987747473));
#53695=CARTESIAN_POINT('Ctrl Pts',(16.1993817363336,-19.3115973546745,-15.4154551936426));
#53696=CARTESIAN_POINT('Ctrl Pts',(16.1860549755609,-19.2176638181479,-15.4201782651282));
#53697=CARTESIAN_POINT('Ctrl Pts',(16.1779317634136,-19.1228307363238,-15.4249013366138));
#53698=CARTESIAN_POINT('Ctrl Pts',(16.1751178968034,-19.0276464271479,-15.4296244080995));
#53699=CARTESIAN_POINT('Ctrl Pts',(16.1743899245164,-19.0030214008619,-15.4308463086469));
#53700=CARTESIAN_POINT('Ctrl Pts',(16.1740170525925,-18.9783729560401,-15.4320682091942));
#53701=CARTESIAN_POINT('Ctrl Pts',(16.174000571626,-18.9537107672549,-15.4332901097416));
#53702=CARTESIAN_POINT('Ctrl Pts',(16.1740005716256,-18.9537107666516,-15.4332901097715));
#53703=CARTESIAN_POINT('Ctrl Pts',(16.1739440307447,-18.8691027211111,-15.437482057942));
#53704=CARTESIAN_POINT('Ctrl Pts',(16.1780862675835,-18.7844696898645,-15.4416740061124));
#53705=CARTESIAN_POINT('Ctrl Pts',(16.1864081330308,-18.7002547332075,-15.4458659542829));
#53706=CARTESIAN_POINT('Ctrl Pts',(16.1947304086796,-18.6160356254258,-15.4500581090829));
#53707=CARTESIAN_POINT('Ctrl Pts',(16.2072326772703,-18.5322350838834,-15.4542502638829));
#53708=CARTESIAN_POINT('Ctrl Pts',(16.2238439368849,-18.4492908009531,-15.4584424186829));
#53709=CARTESIAN_POINT('Ctrl Pts',(16.2404607969944,-18.3663185533138,-15.4626359868701));
#53710=CARTESIAN_POINT('Ctrl Pts',(16.2611893110379,-18.2842035816671,-15.4668295550574));
#53711=CARTESIAN_POINT('Ctrl Pts',(16.2859076895265,-18.2033718951305,-15.4710231232446));
#53712=CARTESIAN_POINT('Ctrl Pts',(16.3106584247114,-18.122434398808,-15.4752221808701));
#53713=CARTESIAN_POINT('Ctrl Pts',(16.3394093150966,-18.0427839738199,-15.4794212384956));
#53714=CARTESIAN_POINT('Ctrl Pts',(16.3719892689075,-17.9648296468169,-15.4836202961211));
#53715=CARTESIAN_POINT('Ctrl Pts',(16.4045936038559,-17.8868169828627,-15.4878224961022));
#53716=CARTESIAN_POINT('Ctrl Pts',(16.4410325111314,-17.8105033515335,-15.4920246960833));
#53717=CARTESIAN_POINT('Ctrl Pts',(16.4810885578785,-17.7362738655611,-15.4962268960645));
#53718=CARTESIAN_POINT('Ctrl Pts',(16.5212156880346,-17.6619126520384,-15.5004365532643));
#53719=CARTESIAN_POINT('Ctrl Pts',(16.5649725361192,-17.5896433529152,-15.5046462104641));
#53720=CARTESIAN_POINT('Ctrl Pts',(16.612098119287,-17.5198224940229,-15.5088558676639));
#53721=CARTESIAN_POINT('Ctrl Pts',(16.6314200308983,-17.4911953158863,-15.5105818648582));
#53722=CARTESIAN_POINT('Ctrl Pts',(16.6513077816386,-17.4629793510679,-15.5123078620525));
#53723=CARTESIAN_POINT('Ctrl Pts',(16.6717415022699,-17.4351974787271,-15.5140338592469));
#53724=CARTESIAN_POINT('Ctrl Pts',(16.7212825156696,-17.3678410665133,-15.5182184936399));
#53725=CARTESIAN_POINT('Ctrl Pts',(16.7742191330187,-17.3027889832897,-15.522403128033));
#53726=CARTESIAN_POINT('Ctrl Pts',(16.8303093008605,-17.2404037502934,-15.526587762426));
#53727=CARTESIAN_POINT('Ctrl Pts',(16.8863196312909,-17.1781073149545,-15.53076644051));
#53728=CARTESIAN_POINT('Ctrl Pts',(16.9454742913219,-17.1184705290969,-15.5349451185939));
#53729=CARTESIAN_POINT('Ctrl Pts',(17.0074891937055,-17.0618252896231,-15.5391237966778));
#53730=CARTESIAN_POINT('Ctrl Pts',(17.070615668645,-17.004164724942,-15.5433773745633));
#53731=CARTESIAN_POINT('Ctrl Pts',(17.1367056485332,-16.949604396855,-15.5476309524487));
#53732=CARTESIAN_POINT('Ctrl Pts',(17.2054179892121,-16.8984574422974,-15.5518845303342));
#53733=CARTESIAN_POINT('Ctrl Pts',(17.272798207086,-16.8483020712589,-15.5560556443121));
#53734=CARTESIAN_POINT('Ctrl Pts',(17.3426996279386,-16.8014291923403,-15.5602267582901));
#53735=CARTESIAN_POINT('Ctrl Pts',(17.4147663076937,-16.7580942442566,-15.564397872268));
#53736=CARTESIAN_POINT('Ctrl Pts',(17.4868088047782,-16.7147738376334,-15.5685675865884));
#53737=CARTESIAN_POINT('Ctrl Pts',(17.5610147238611,-16.6749892409427,-15.5727373009088));
#53738=CARTESIAN_POINT('Ctrl Pts',(17.6370000578042,-16.6389519834594,-15.5769070152291));
#53739=CARTESIAN_POINT('Ctrl Pts',(17.7129826878631,-16.6029160083363,-15.5810765811732));
#53740=CARTESIAN_POINT('Ctrl Pts',(17.7907441908668,-16.570627303655,-15.5852461471172));
#53741=CARTESIAN_POINT('Ctrl Pts',(17.8698781766138,-16.5422503295264,-15.5894157130613));
#53742=CARTESIAN_POINT('Ctrl Pts',(17.9517944156772,-16.5128756559942,-15.5937318758002));
#53743=CARTESIAN_POINT('Ctrl Pts',(18.0351809497174,-16.4876930819298,-15.5980480385391));
#53744=CARTESIAN_POINT('Ctrl Pts',(18.1195690084032,-16.4668290689441,-15.602364201278));
#53745=CARTESIAN_POINT('Ctrl Pts',(18.2012081349535,-16.4466446989869,-15.6065397654697));
#53746=CARTESIAN_POINT('Ctrl Pts',(18.28378406749,-16.4305019005906,-15.6107153296614));
#53747=CARTESIAN_POINT('Ctrl Pts',(18.3668630221885,-16.4184628600466,-15.6148908938531));
#53748=CARTESIAN_POINT('Ctrl Pts',(18.4541380973873,-16.4058157561847,-15.6192773558656));
#53749=CARTESIAN_POINT('Ctrl Pts',(18.541967764093,-16.3976979204099,-15.6236638178782));
#53750=CARTESIAN_POINT('Ctrl Pts',(18.6298465962986,-16.3941196141146,-15.6280502798907));
#53751=CARTESIAN_POINT('Ctrl Pts',(18.7177254285043,-16.3905413078192,-15.6324367419032));
#53752=CARTESIAN_POINT('Ctrl Pts',(18.8056528468588,-16.391502448601,-15.6368232039158));
#53753=CARTESIAN_POINT('Ctrl Pts',(18.8931294701919,-16.3969505265619,-15.6412096659283));
#53754=CARTESIAN_POINT('Ctrl Pts',(18.9765715593007,-16.4021473321696,-15.6453938186788));
#53755=CARTESIAN_POINT('Ctrl Pts',(19.059914071307,-16.4114456475973,-15.6495779714293));
#53756=CARTESIAN_POINT('Ctrl Pts',(19.1427213148447,-16.4248381755828,-15.6537621241798));
#53757=CARTESIAN_POINT('Ctrl Pts',(19.2254168838738,-16.4382126422983,-15.6579406341485));
#53758=CARTESIAN_POINT('Ctrl Pts',(19.3075781677335,-16.4556702853466,-15.6621191441173));
#53759=CARTESIAN_POINT('Ctrl Pts',(19.3887723742188,-16.4771518959823,-15.666297654086));
#53760=CARTESIAN_POINT('Ctrl Pts',(19.4703186695032,-16.4987266590094,-15.6704942836549));
#53761=CARTESIAN_POINT('Ctrl Pts',(19.5508890109359,-16.5243603457589,-15.6746909132238));
#53762=CARTESIAN_POINT('Ctrl Pts',(19.630053111369,-16.5539406134113,-15.6788875427928));
#53763=CARTESIAN_POINT('Ctrl Pts',(19.7087329159883,-16.5833399202531,-15.6830584989804));
#53764=CARTESIAN_POINT('Ctrl Pts',(19.7860232004139,-16.6166374960991,-15.6872294551681));
#53765=CARTESIAN_POINT('Ctrl Pts',(19.8615163112604,-16.653673006763,-15.6914004113557));
#53766=CARTESIAN_POINT('Ctrl Pts',(19.937706443364,-16.6910504630417,-15.6956098776153));
#53767=CARTESIAN_POINT('Ctrl Pts',(20.0120655925479,-16.7322350830384,-15.6998193438748));
#53768=CARTESIAN_POINT('Ctrl Pts',(20.0841966779277,-16.7770128894835,-15.7040288101343));
#53769=CARTESIAN_POINT('Ctrl Pts',(20.1563277633076,-16.8217906959285,-15.7082382763939));
#53770=CARTESIAN_POINT('Ctrl Pts',(20.2262303743025,-16.8701614355123,-15.7124477426534));
#53771=CARTESIAN_POINT('Ctrl Pts',(20.293535888361,-16.9218650751948,-15.7166572089129));
#53772=CARTESIAN_POINT('',(16.1740008768645,-18.949881145288,-15.3667098902285));
#53773=CARTESIAN_POINT('Ctrl Pts',(16.1723624843679,-18.9498797892267,-15.3667098902285));
#53774=CARTESIAN_POINT('Ctrl Pts',(16.1710770695818,-18.8056440598866,-15.3738974629702));
#53775=CARTESIAN_POINT('Ctrl Pts',(16.2478506876061,-17.8120819459935,-15.4234769712724));
#53776=CARTESIAN_POINT('Ctrl Pts',(17.5479306946412,-16.1669449835732,-15.515448415135));
#53777=CARTESIAN_POINT('Ctrl Pts',(19.5288321013839,-16.3593204888311,-15.6027438735347));
#53778=CARTESIAN_POINT('Ctrl Pts',(20.2561600515754,-16.8880018374306,-15.6476473963739));
#53779=CARTESIAN_POINT('Ctrl Pts',(20.295887153474,-16.918834963786,-15.6501589836526));
#53780=CARTESIAN_POINT('Ctrl Pts',(20.2935358883611,-16.9218650751948,-14.8500370296196));
#53781=CARTESIAN_POINT('Ctrl Pts',(20.360176577277,-16.9730580007091,-14.8542147193799));
#53782=CARTESIAN_POINT('Ctrl Pts',(20.4242278292755,-17.0274848208923,-14.8583924091402));
#53783=CARTESIAN_POINT('Ctrl Pts',(20.4853757399687,-17.0848409233681,-14.8625700989005));
#53784=CARTESIAN_POINT('Ctrl Pts',(20.5466225444612,-17.1422897871961,-14.8667545451895));
#53785=CARTESIAN_POINT('Ctrl Pts',(20.6049563187768,-17.2026770568638,-14.8709389914784));
#53786=CARTESIAN_POINT('Ctrl Pts',(20.6601019172694,-17.2656633182276,-14.8751234377674));
#53787=CARTESIAN_POINT('Ctrl Pts',(20.6796325173081,-17.2879708008238,-14.8766054190876));
#53788=CARTESIAN_POINT('Ctrl Pts',(20.6987636051395,-17.3106040028926,-14.8780874004077));
#53789=CARTESIAN_POINT('Ctrl Pts',(20.7174842649081,-17.3335469821889,-14.8795693817278));
#53790=CARTESIAN_POINT('Ctrl Pts',(20.770345333846,-17.398330511467,-14.8837540161209));
#53791=CARTESIAN_POINT('Ctrl Pts',(20.8201275486196,-17.4658271045687,-14.8879386505139));
#53792=CARTESIAN_POINT('Ctrl Pts',(20.866540268707,-17.5357118928893,-14.892123284907));
#53793=CARTESIAN_POINT('Ctrl Pts',(20.912886926032,-17.6054972088638,-14.8963019629909));
#53794=CARTESIAN_POINT('Ctrl Pts',(20.9558733628219,-17.6776635880367,-14.9004806410749));
#53795=CARTESIAN_POINT('Ctrl Pts',(20.9952490842181,-17.7518531010236,-14.9046593191588));
#53796=CARTESIAN_POINT('Ctrl Pts',(21.0353305871216,-17.8273724077117,-14.9089128970442));
#53797=CARTESIAN_POINT('Ctrl Pts',(21.0716703524657,-17.9049877173955,-14.9131664749297));
#53798=CARTESIAN_POINT('Ctrl Pts',(21.1040502914402,-17.9842905311798,-14.9174200528151));
#53799=CARTESIAN_POINT('Ctrl Pts',(21.1358024821134,-18.0620559051722,-14.9215911667931));
#53800=CARTESIAN_POINT('Ctrl Pts',(21.1637468322872,-18.1414434905285,-14.925762280771));
#53801=CARTESIAN_POINT('Ctrl Pts',(21.1877248192283,-18.222044856513,-14.929933394749));
#53802=CARTESIAN_POINT('Ctrl Pts',(21.2116947601243,-18.3026191759308,-14.9341031090694));
#53803=CARTESIAN_POINT('Ctrl Pts',(21.2317008500143,-18.3844060265126,-14.9382728233897));
#53804=CARTESIAN_POINT('Ctrl Pts',(21.2476340898709,-18.46698076096,-14.9424425377101));
#53805=CARTESIAN_POINT('Ctrl Pts',(21.2635667627544,-18.5495525570439,-14.9466121036542));
#53806=CARTESIAN_POINT('Ctrl Pts',(21.2754267874402,-18.6329117293876,-14.9507816695982));
#53807=CARTESIAN_POINT('Ctrl Pts',(21.2831563307877,-18.7166237029669,-14.9549512355422));
#53808=CARTESIAN_POINT('Ctrl Pts',(21.2911576353439,-18.8032788862672,-14.9592673982812));
#53809=CARTESIAN_POINT('Ctrl Pts',(21.2947325504218,-18.8903116161907,-14.9635835610201));
#53810=CARTESIAN_POINT('Ctrl Pts',(21.2938756072079,-18.9772363947924,-14.967899723759));
#53811=CARTESIAN_POINT('Ctrl Pts',(21.293046578829,-19.0613296078741,-14.9720752879507));
#53812=CARTESIAN_POINT('Ctrl Pts',(21.2880700686645,-19.1453213272334,-14.9762508521424));
#53813=CARTESIAN_POINT('Ctrl Pts',(21.2789941177451,-19.2287759755517,-14.9804264163341));
#53814=CARTESIAN_POINT('Ctrl Pts',(21.2694597621209,-19.3164457197619,-14.9848128783466));
#53815=CARTESIAN_POINT('Ctrl Pts',(21.2554010498833,-19.4035221357511,-14.9891993403591));
#53816=CARTESIAN_POINT('Ctrl Pts',(21.2369341836446,-19.4895132299242,-14.9935858023717));
#53817=CARTESIAN_POINT('Ctrl Pts',(21.2184673174058,-19.5755043240972,-14.9979722643842));
#53818=CARTESIAN_POINT('Ctrl Pts',(21.1955925215497,-19.6604095560011,-15.0023587263967));
#53819=CARTESIAN_POINT('Ctrl Pts',(21.1684852750765,-19.7437584514458,-15.0067451884093));
#53820=CARTESIAN_POINT('Ctrl Pts',(21.142625273196,-19.8232723406584,-15.0109298228023));
#53821=CARTESIAN_POINT('Ctrl Pts',(21.1128174886275,-19.9016659307485,-15.0151144571954));
#53822=CARTESIAN_POINT('Ctrl Pts',(21.0791777662538,-19.9785189938178,-15.0192990915884));
#53823=CARTESIAN_POINT('Ctrl Pts',(21.0455859258611,-20.0552626660644,-15.0234777696724));
#53824=CARTESIAN_POINT('Ctrl Pts',(21.0081731644859,-20.1304697489562,-15.0276564477563));
#53825=CARTESIAN_POINT('Ctrl Pts',(20.9671048559811,-20.2037358755718,-15.0318351258403));
#53826=CARTESIAN_POINT('Ctrl Pts',(20.9253004275616,-20.2783152448517,-15.0360887037257));
#53827=CARTESIAN_POINT('Ctrl Pts',(20.8797082607492,-20.3508829316546,-15.0403422816111));
#53828=CARTESIAN_POINT('Ctrl Pts',(20.8305537911317,-20.4210344451004,-15.0445958594966));
#53829=CARTESIAN_POINT('Ctrl Pts',(20.7823522768248,-20.4898259345685,-15.0487669734745));
#53830=CARTESIAN_POINT('Ctrl Pts',(20.7307256276405,-20.5562937050241,-15.0529380874525));
#53831=CARTESIAN_POINT('Ctrl Pts',(20.675931463843,-20.6200833881244,-15.0571092014304));
#53832=CARTESIAN_POINT('Ctrl Pts',(20.6211556867563,-20.6838516659805,-15.0612789157508));
#53833=CARTESIAN_POINT('Ctrl Pts',(20.5632148054787,-20.7449432925553,-15.0654486300712));
#53834=CARTESIAN_POINT('Ctrl Pts',(20.5024068820801,-20.8030367633874,-15.0696183443915));
#53835=CARTESIAN_POINT('Ctrl Pts',(20.4416011224884,-20.8611281670045,-15.0737879103356));
#53836=CARTESIAN_POINT('Ctrl Pts',(20.3779288568417,-20.9162213098335,-15.0779574762796));
#53837=CARTESIAN_POINT('Ctrl Pts',(20.3117241899802,-20.9680323361373,-15.0821270422237));
#53838=CARTESIAN_POINT('Ctrl Pts',(20.2431918487041,-21.0216649742102,-15.0864432049626));
#53839=CARTESIAN_POINT('Ctrl Pts',(20.1719461297946,-21.0717800780495,-15.0907593677015));
#53840=CARTESIAN_POINT('Ctrl Pts',(20.0983923000264,-21.1181102584191,-15.0950755304404));
#53841=CARTESIAN_POINT('Ctrl Pts',(20.0272344785266,-21.1629312380363,-15.0992510946321));
#53842=CARTESIAN_POINT('Ctrl Pts',(19.9539170439582,-21.2042099051979,-15.1034266588238));
#53843=CARTESIAN_POINT('Ctrl Pts',(19.8788322516134,-21.2417508850672,-15.1076022230155));
#53844=CARTESIAN_POINT('Ctrl Pts',(19.7999551049042,-21.2811879705845,-15.111988685028));
#53845=CARTESIAN_POINT('Ctrl Pts',(19.7191279049091,-21.3164996308723,-15.1163751470406));
#53846=CARTESIAN_POINT('Ctrl Pts',(19.6368272386519,-21.3475172671363,-15.1207616090531));
#53847=CARTESIAN_POINT('Ctrl Pts',(19.5545265723946,-21.3785349034004,-15.1251480710657));
#53848=CARTESIAN_POINT('Ctrl Pts',(19.4707530157655,-21.4052584117748,-15.1295345330782));
#53849=CARTESIAN_POINT('Ctrl Pts',(19.3859971465586,-21.4275806835729,-15.1339209950908));
#53850=CARTESIAN_POINT('Ctrl Pts',(19.3051410205324,-21.4488758745561,-15.1381056294838));
#53851=CARTESIAN_POINT('Ctrl Pts',(19.2230900288836,-21.4662452083819,-15.1422902638769));
#53852=CARTESIAN_POINT('Ctrl Pts',(19.1402602214101,-21.4795586308728,-15.1464748982699));
#53853=CARTESIAN_POINT('Ctrl Pts',(19.0575483119153,-21.4928531033548,-15.1506535763538));
#53854=CARTESIAN_POINT('Ctrl Pts',(18.974060238839,-21.5021030592902,-15.1548322544378));
#53855=CARTESIAN_POINT('Ctrl Pts',(18.8902255244996,-21.5072286757734,-15.1590109325217));
#53856=CARTESIAN_POINT('Ctrl Pts',(18.8048881331567,-21.5124461652484,-15.1632645104072));
#53857=CARTESIAN_POINT('Ctrl Pts',(18.7191920174691,-21.5133898805874,-15.1675180882926));
#53858=CARTESIAN_POINT('Ctrl Pts',(18.6335993142633,-21.510030434202,-15.171771666178));
#53859=CARTESIAN_POINT('Ctrl Pts',(18.5496659926296,-21.5067361172402,-15.175942780156));
#53860=CARTESIAN_POINT('Ctrl Pts',(18.4658325904026,-21.4993040188572,-15.1801138941339));
#53861=CARTESIAN_POINT('Ctrl Pts',(18.3825365202413,-21.4877589440631,-15.1842850081119));
#53862=CARTESIAN_POINT('Ctrl Pts',(18.2992684008808,-21.4762177433303,-15.1884547224323));
#53863=CARTESIAN_POINT('Ctrl Pts',(18.2165377107911,-21.4605663702896,-15.1926244367526));
#53864=CARTESIAN_POINT('Ctrl Pts',(18.1347761196902,-21.4408814237055,-15.196794151073));
#53865=CARTESIAN_POINT('Ctrl Pts',(18.0530174380175,-21.4211971775963,-15.200963717017));
#53866=CARTESIAN_POINT('Ctrl Pts',(17.9722282338226,-21.3974797518311,-15.2051332829611));
#53867=CARTESIAN_POINT('Ctrl Pts',(17.8928280294726,-21.3698564299807,-15.2093028489051));
#53868=CARTESIAN_POINT('Ctrl Pts',(17.8106362118883,-21.3412619062111,-15.213619011644));
#53869=CARTESIAN_POINT('Ctrl Pts',(17.729933384083,-21.3084818866878,-15.217935174383));
#53870=CARTESIAN_POINT('Ctrl Pts',(17.6511637413075,-21.2717124039115,-15.2222513371219));
#53871=CARTESIAN_POINT('Ctrl Pts',(17.5749600113602,-21.2361406831691,-15.2264269013136));
#53872=CARTESIAN_POINT('Ctrl Pts',(17.5005658480113,-21.1968356830554,-15.2306024655052));
#53873=CARTESIAN_POINT('Ctrl Pts',(17.4283578509295,-21.1540214755017,-15.2347780296969));
#53874=CARTESIAN_POINT('Ctrl Pts',(17.3525027995735,-21.1090448241056,-15.2391644917095));
#53875=CARTESIAN_POINT('Ctrl Pts',(17.2790610511148,-21.0601954720667,-15.243550953722));
#53876=CARTESIAN_POINT('Ctrl Pts',(17.2084323379748,-21.007782894321,-15.2479374157345));
#53877=CARTESIAN_POINT('Ctrl Pts',(17.1378036248349,-20.9553703165754,-15.252323877747));
#53878=CARTESIAN_POINT('Ctrl Pts',(17.0699883460669,-20.8993949411349,-15.2567103397596));
#53879=CARTESIAN_POINT('Ctrl Pts',(17.0053421035814,-20.8402112903883,-15.2610968017721));
#53880=CARTESIAN_POINT('Ctrl Pts',(16.9445899812057,-20.7845927075508,-15.2652190348167));
#53881=CARTESIAN_POINT('Ctrl Pts',(16.8863955977248,-20.7259204795934,-15.2693412678613));
#53882=CARTESIAN_POINT('Ctrl Pts',(16.8310887538618,-20.6644627847987,-15.2734635009059));
#53883=CARTESIAN_POINT('Ctrl Pts',(16.7758743514522,-20.6031078121671,-15.2775788439313));
#53884=CARTESIAN_POINT('Ctrl Pts',(16.7235382140149,-20.5389769727691,-15.2816941869567));
#53885=CARTESIAN_POINT('Ctrl Pts',(16.6743754759298,-20.4723771965696,-15.2858095299821));
#53886=CARTESIAN_POINT('Ctrl Pts',(16.6252589923643,-20.4058400804408,-15.2899210011073));
#53887=CARTESIAN_POINT('Ctrl Pts',(16.5793102664141,-20.336839014796,-15.2940324722326));
#53888=CARTESIAN_POINT('Ctrl Pts',(16.5367853878613,-20.2657153223604,-15.2981439433578));
#53889=CARTESIAN_POINT('Ctrl Pts',(16.4942868717937,-20.1946357216976,-15.3022528656552));
#53890=CARTESIAN_POINT('Ctrl Pts',(16.4552082342186,-20.1214365120742,-15.3063617879525));
#53891=CARTESIAN_POINT('Ctrl Pts',(16.4197623875945,-20.0464881330228,-15.3104707102498));
#53892=CARTESIAN_POINT('Ctrl Pts',(16.3843271437787,-19.971562173052,-15.3145784034577));
#53893=CARTESIAN_POINT('Ctrl Pts',(16.3525227351499,-19.894888512104,-15.3186860966657));
#53894=CARTESIAN_POINT('Ctrl Pts',(16.3245154961056,-19.8168609284116,-15.3227937898736));
#53895=CARTESIAN_POINT('Ctrl Pts',(16.2964946934766,-19.7387955568548,-15.3269034723902));
#53896=CARTESIAN_POINT('Ctrl Pts',(16.272274898332,-19.6593753990486,-15.3310131549069));
#53897=CARTESIAN_POINT('Ctrl Pts',(16.2519734104534,-19.5790119686126,-15.3351228374235));
#53898=CARTESIAN_POINT('Ctrl Pts',(16.231666738396,-19.4986280166076,-15.3392335693868));
#53899=CARTESIAN_POINT('Ctrl Pts',(16.2152804642378,-19.4173007774467,-15.3433443013501));
#53900=CARTESIAN_POINT('Ctrl Pts',(16.2028808242122,-19.3354523672626,-15.3474550333134));
#53901=CARTESIAN_POINT('Ctrl Pts',(16.1904661338132,-19.2535046115225,-15.3515707547805));
#53902=CARTESIAN_POINT('Ctrl Pts',(16.1820477886731,-19.1710348943536,-15.3556864762476));
#53903=CARTESIAN_POINT('Ctrl Pts',(16.1776401048971,-19.0884700945614,-15.3598021977147));
#53904=CARTESIAN_POINT('Ctrl Pts',(16.1751742007241,-19.04227873994,-15.362104761886));
#53905=CARTESIAN_POINT('Ctrl Pts',(16.173962657598,-18.9960576424388,-15.3644073260572));
#53906=CARTESIAN_POINT('Ctrl Pts',(16.1740008768645,-18.949881145288,-15.3667098902285));
#53907=CARTESIAN_POINT('Origin',(18.734,-18.952,1.76670989022851));
#53908=CARTESIAN_POINT('',(20.2909850430174,-16.9251769135511,-14.0501277865439));
#53909=CARTESIAN_POINT('',(20.2961055948522,-16.9185282149957,-14.1167030459603));
#53910=CARTESIAN_POINT('',(20.293535888361,-16.9218650751948,1.76670989022851));
#53911=CARTESIAN_POINT('',(16.1738766836434,-18.9531301832654,-14.6332901097715));
#53912=CARTESIAN_POINT('Ctrl Pts',(20.2961055948522,-16.9185282149957,-14.1167030459603));
#53913=CARTESIAN_POINT('Ctrl Pts',(20.959851318088,-17.429684584912,-14.1585606281177));
#53914=CARTESIAN_POINT('Ctrl Pts',(21.7469835062583,-19.1757114502307,-14.2428101458356));
#53915=CARTESIAN_POINT('Ctrl Pts',(20.1889474246921,-21.6065091003007,-14.369451599114));
#53916=CARTESIAN_POINT('Ctrl Pts',(17.2895133775451,-21.6122159629899,-14.4966274057954));
#53917=CARTESIAN_POINT('Ctrl Pts',(16.2008983314107,-19.9284205945985,-14.5845735760146));
#53918=CARTESIAN_POINT('Ctrl Pts',(16.1700292378907,-19.0164624118087,-14.6301278106733));
#53919=CARTESIAN_POINT('Ctrl Pts',(16.1703790167221,-18.9531317273334,-14.6332901097715));
#53920=CARTESIAN_POINT('Ctrl Pts',(16.1740002494514,-18.9531301287164,-14.6332901097715));
#53921=CARTESIAN_POINT('Ctrl Pts',(16.1739637014967,-18.8703406609987,-14.6374299052976));
#53922=CARTESIAN_POINT('Ctrl Pts',(16.1779474618949,-18.787387492894,-14.6415697008237));
#53923=CARTESIAN_POINT('Ctrl Pts',(16.1859729132155,-18.7046986352396,-14.6457094963498));
#53924=CARTESIAN_POINT('Ctrl Pts',(16.1939875490477,-18.6221212131097,-14.6498437128863));
#53925=CARTESIAN_POINT('Ctrl Pts',(16.2060330170348,-18.5398078587028,-14.6539779294227));
#53926=CARTESIAN_POINT('Ctrl Pts',(16.2220786798974,-18.4581869973217,-14.6581121459591));
#53927=CARTESIAN_POINT('Ctrl Pts',(16.2381078732803,-18.3766499126678,-14.6622421190812));
#53928=CARTESIAN_POINT('Ctrl Pts',(16.2581290152451,-18.2958043686403,-14.6663720922033));
#53929=CARTESIAN_POINT('Ctrl Pts',(16.2820597821146,-18.2160725797227,-14.6705020653254));
#53930=CARTESIAN_POINT('Ctrl Pts',(16.3059775967093,-18.1363839447938,-14.6746298031431));
#53931=CARTESIAN_POINT('Ctrl Pts',(16.3338007023324,-18.0578083185529,-14.6787575409609));
#53932=CARTESIAN_POINT('Ctrl Pts',(16.3653962152435,-17.9807553805363,-14.6828852787787));
#53933=CARTESIAN_POINT('Ctrl Pts',(16.3969845852848,-17.9037198620533,-14.6870120834293));
#53934=CARTESIAN_POINT('Ctrl Pts',(16.4323434905918,-17.8282067834232,-14.69113888808));
#53935=CARTESIAN_POINT('Ctrl Pts',(16.4712914723378,-17.7546069488907,-14.6952656927306));
#53936=CARTESIAN_POINT('Ctrl Pts',(16.510242924153,-17.6810005569833,-14.6993928650588));
#53937=CARTESIAN_POINT('Ctrl Pts',(16.5527838651356,-17.609308162424,-14.703520037387));
#53938=CARTESIAN_POINT('Ctrl Pts',(16.5986870593953,-17.5398956675635,-14.7076472097152));
#53939=CARTESIAN_POINT('Ctrl Pts',(16.6446377721095,-17.4704113176929,-14.7117786544443));
#53940=CARTESIAN_POINT('Ctrl Pts',(16.6939574240315,-17.4032119705958,-14.7159100991734));
#53941=CARTESIAN_POINT('Ctrl Pts',(16.746376041612,-17.3386336435756,-14.7200415439026));
#53942=CARTESIAN_POINT('Ctrl Pts',(16.7988250781874,-17.2740178411719,-14.7241753861462));
#53943=CARTESIAN_POINT('Ctrl Pts',(16.8543763437697,-17.2120264344659,-14.7283092283899));
#53944=CARTESIAN_POINT('Ctrl Pts',(16.9127219511753,-17.1529596255589,-14.7324430706335));
#53945=CARTESIAN_POINT('Ctrl Pts',(16.9711635405876,-17.0937956482256,-14.7365837132944));
#53946=CARTESIAN_POINT('Ctrl Pts',(17.0324082986517,-17.0375661867597,-14.7407243559553));
#53947=CARTESIAN_POINT('Ctrl Pts',(17.0961145829386,-16.9845317383557,-14.7448649986161));
#53948=CARTESIAN_POINT('Ctrl Pts',(17.1274705472736,-16.9584284066154,-14.7469030054635));
#53949=CARTESIAN_POINT('Ctrl Pts',(17.1594223751532,-16.9330984310461,-14.7489410123109));
#53950=CARTESIAN_POINT('Ctrl Pts',(17.1919269101816,-16.9085689182999,-14.7509790191583));
#53951=CARTESIAN_POINT('Ctrl Pts',(17.2586683911458,-16.8582025307613,-14.7551636535514));
#53952=CARTESIAN_POINT('Ctrl Pts',(17.3280042311001,-16.8110156651531,-14.7593482879444));
#53953=CARTESIAN_POINT('Ctrl Pts',(17.3995987737075,-16.767286433587,-14.7635329223375));
#53954=CARTESIAN_POINT('Ctrl Pts',(17.4710914103451,-16.7236194451695,-14.7677116004214));
#53955=CARTESIAN_POINT('Ctrl Pts',(17.5448359744308,-16.6834005528598,-14.7718902785053));
#53956=CARTESIAN_POINT('Ctrl Pts',(17.6204652949934,-16.6468664982813,-14.7760689565893));
#53957=CARTESIAN_POINT('Ctrl Pts',(17.6974502167732,-16.6096775970311,-14.7803225344747));
#53958=CARTESIAN_POINT('Ctrl Pts',(17.7763877432994,-16.5763072247155,-14.7845761123602));
#53959=CARTESIAN_POINT('Ctrl Pts',(17.8568613993349,-16.5469578225687,-14.7888296902456));
#53960=CARTESIAN_POINT('Ctrl Pts',(17.9357749165169,-16.5181774158532,-14.7930008042235));
#53961=CARTESIAN_POINT('Ctrl Pts',(18.0161650809,-16.4932636267837,-14.7971719182015));
#53962=CARTESIAN_POINT('Ctrl Pts',(18.0976177441666,-16.4723593759457,-14.8013430321794));
#53963=CARTESIAN_POINT('Ctrl Pts',(18.1790430752053,-16.451462139731,-14.8055127464998));
#53964=CARTESIAN_POINT('Ctrl Pts',(18.2615297518284,-16.434571883947,-14.8096824608202));
#53965=CARTESIAN_POINT('Ctrl Pts',(18.3446492988108,-16.4217814261445,-14.8138521751405));
#53966=CARTESIAN_POINT('Ctrl Pts',(18.4277658880431,-16.4089914234813,-14.8180217410846));
#53967=CARTESIAN_POINT('Ctrl Pts',(18.5115148480479,-16.4003009978601,-14.8221913070286));
#53968=CARTESIAN_POINT('Ctrl Pts',(18.5954597232801,-16.3957514612764,-14.8263608729727));
#53969=CARTESIAN_POINT('Ctrl Pts',(18.6823559967683,-16.3910419685989,-14.8306770357116));
#53970=CARTESIAN_POINT('Ctrl Pts',(18.7694616919212,-16.3907699986349,-14.8349931984505));
#53971=CARTESIAN_POINT('Ctrl Pts',(18.8562914526112,-16.3949226056652,-14.8393093611894));
#53972=CARTESIAN_POINT('Ctrl Pts',(18.9402927429795,-16.3989399419582,-14.8434849253811));
#53973=CARTESIAN_POINT('Ctrl Pts',(19.0240353356995,-16.4070979281598,-14.8476604895728));
#53974=CARTESIAN_POINT('Ctrl Pts',(19.1070857885139,-16.4193320402372,-14.8518360537645));
#53975=CARTESIAN_POINT('Ctrl Pts',(19.1943309222662,-16.4321840682319,-14.856222515777));
#53976=CARTESIAN_POINT('Ctrl Pts',(19.2808115861347,-16.4495346990029,-14.8606089777895));
#53977=CARTESIAN_POINT('Ctrl Pts',(19.3660405469235,-16.471249156597,-14.8649954398021));
#53978=CARTESIAN_POINT('Ctrl Pts',(19.4512695077123,-16.4929636141912,-14.8693819018146));
#53979=CARTESIAN_POINT('Ctrl Pts',(19.5352462338659,-16.5190416538915,-14.8737683638271));
#53980=CARTESIAN_POINT('Ctrl Pts',(19.6175072439393,-16.549290082031,-14.8781548258396));
#53981=CARTESIAN_POINT('Ctrl Pts',(19.6959730538366,-16.5781429664043,-14.8823389137093));
#53982=CARTESIAN_POINT('Ctrl Pts',(19.7731699980655,-16.6108972906671,-14.886523001579));
#53983=CARTESIAN_POINT('Ctrl Pts',(19.8486827058591,-16.6474214126529,-14.8907070894487));
#53984=CARTESIAN_POINT('Ctrl Pts',(19.9270438220701,-16.6853232579325,-14.8950490049405));
#53985=CARTESIAN_POINT('Ctrl Pts',(20.0035906250348,-16.7272848683664,-14.8993909204323));
#53986=CARTESIAN_POINT('Ctrl Pts',(20.0778772798292,-16.7731026052706,-14.9037328359241));
#53987=CARTESIAN_POINT('Ctrl Pts',(20.1521639346237,-16.8189203421747,-14.9080747514158));
#53988=CARTESIAN_POINT('Ctrl Pts',(20.2241899296921,-16.8685939797933,-14.9124166669076));
#53989=CARTESIAN_POINT('Ctrl Pts',(20.293535888361,-16.9218650751948,-14.9167585823994));
#53990=CARTESIAN_POINT('',(16.1743645121285,-18.9514398261319,-14.566709915053));
#53991=CARTESIAN_POINT('Ctrl Pts',(16.1740000613162,-18.9514396975223,-14.5667099174731));
#53992=CARTESIAN_POINT('Ctrl Pts',(16.1740197372988,-18.8615409084374,-14.571157199272));
#53993=CARTESIAN_POINT('Ctrl Pts',(16.1787790795978,-18.7717655181971,-14.575604481071));
#53994=CARTESIAN_POINT('Ctrl Pts',(16.1882138900512,-18.6826060832318,-14.58005176287));
#53995=CARTESIAN_POINT('Ctrl Pts',(16.1976832329536,-18.5931203148802,-14.5845153222119));
#53996=CARTESIAN_POINT('Ctrl Pts',(16.211862232535,-18.504255369482,-14.5889788815538));
#53997=CARTESIAN_POINT('Ctrl Pts',(16.23063522025,-18.4164957707849,-14.5934424408956));
#53998=CARTESIAN_POINT('Ctrl Pts',(16.2494446598934,-18.3285657673207,-14.5979146672301));
#53999=CARTESIAN_POINT('Ctrl Pts',(16.2728657964755,-18.241745739755,-14.6023868935646));
#54000=CARTESIAN_POINT('Ctrl Pts',(16.3007333122773,-18.1565044145825,-14.606859119899));
#54001=CARTESIAN_POINT('Ctrl Pts',(16.3286838403159,-18.0710091710796,-14.6113446681784));
#54002=CARTESIAN_POINT('Ctrl Pts',(16.3611071025136,-17.9871023685302,-14.6158302164579));
#54003=CARTESIAN_POINT('Ctrl Pts',(16.3977895032111,-17.9052333045547,-14.6203157647373));
#54004=CARTESIAN_POINT('Ctrl Pts',(16.4111522146039,-17.8754099382236,-14.6219497659465));
#54005=CARTESIAN_POINT('Ctrl Pts',(16.4250796827618,-17.8458567318514,-14.6235837671557));
#54006=CARTESIAN_POINT('Ctrl Pts',(16.4395601204677,-17.8165945045,-14.625217768365));
#54007=CARTESIAN_POINT('Ctrl Pts',(16.4766441429939,-17.7416547050056,-14.629402402758));
#54008=CARTESIAN_POINT('Ctrl Pts',(16.5174725051856,-17.6683941847451,-14.6335870371511));
#54009=CARTESIAN_POINT('Ctrl Pts',(16.5618698248528,-17.5972120083883,-14.6377716715441));
#54010=CARTESIAN_POINT('Ctrl Pts',(16.6062039504308,-17.526131151049,-14.641950349628));
#54011=CARTESIAN_POINT('Ctrl Pts',(16.6540967016935,-17.4571231485617,-14.646129027712));
#54012=CARTESIAN_POINT('Ctrl Pts',(16.7053259809371,-17.3905642106128,-14.6503077057959));
#54013=CARTESIAN_POINT('Ctrl Pts',(16.7574735081934,-17.3228122515363,-14.6545612836814));
#54014=CARTESIAN_POINT('Ctrl Pts',(16.8130781406444,-17.2575984516733,-14.6588148615668));
#54015=CARTESIAN_POINT('Ctrl Pts',(16.871858331947,-17.1952904599505,-14.6630684394522));
#54016=CARTESIAN_POINT('Ctrl Pts',(16.9294989545411,-17.1341904302313,-14.6672395534302));
#54017=CARTESIAN_POINT('Ctrl Pts',(16.9901927757376,-17.0758848946116,-14.6714106674081));
#54018=CARTESIAN_POINT('Ctrl Pts',(17.0536336491123,-17.0206872529794,-14.6755817813861));
#54019=CARTESIAN_POINT('Ctrl Pts',(17.1170532342893,-16.9655081334488,-14.6797514957065));
#54020=CARTESIAN_POINT('Ctrl Pts',(17.1832176941667,-16.913435138433,-14.6839212100268));
#54021=CARTESIAN_POINT('Ctrl Pts',(17.2517856166925,-16.8647433023425,-14.6880909243472));
#54022=CARTESIAN_POINT('Ctrl Pts',(17.3203510992773,-16.8160531989164,-14.6922604902913));
#54023=CARTESIAN_POINT('Ctrl Pts',(17.3913194988898,-16.7707442808558,-14.6964300562353));
#54024=CARTESIAN_POINT('Ctrl Pts',(17.4643191824367,-16.7290491185112,-14.7005996221793));
#54025=CARTESIAN_POINT('Ctrl Pts',(17.5398854448023,-16.6858880056951,-14.7049157849183));
#54026=CARTESIAN_POINT('Ctrl Pts',(17.6176280306767,-16.6465997576135,-14.7092319476572));
#54027=CARTESIAN_POINT('Ctrl Pts',(17.697107273311,-16.6113903628884,-14.7135481103961));
#54028=CARTESIAN_POINT('Ctrl Pts',(17.7739974879763,-16.5773279104932,-14.7177236745878));
#54029=CARTESIAN_POINT('Ctrl Pts',(17.8525124972024,-16.5470827802973,-14.7218992387795));
#54030=CARTESIAN_POINT('Ctrl Pts',(17.9322359204944,-16.5207915842498,-14.7260748029711));
#54031=CARTESIAN_POINT('Ctrl Pts',(18.0159859843726,-16.4931724823913,-14.7304612649837));
#54032=CARTESIAN_POINT('Ctrl Pts',(18.1010691812454,-16.4699173921692,-14.7348477269962));
#54033=CARTESIAN_POINT('Ctrl Pts',(18.1869895560292,-16.4511242385543,-14.7392341890088));
#54034=CARTESIAN_POINT('Ctrl Pts',(18.272909930813,-16.4323310849394,-14.7436206510213));
#54035=CARTESIAN_POINT('Ctrl Pts',(18.3596668986516,-16.4179998874471,-14.7480071130339));
#54036=CARTESIAN_POINT('Ctrl Pts',(18.446759550604,-16.4081657042506,-14.7523935750464));
#54037=CARTESIAN_POINT('Ctrl Pts',(18.5298216106109,-16.3987866407306,-14.7565770344168));
#54038=CARTESIAN_POINT('Ctrl Pts',(18.6134980569013,-16.3934626556782,-14.7607604937872));
#54039=CARTESIAN_POINT('Ctrl Pts',(18.697358772211,-16.3922622360042,-14.7649439531576));
#54040=CARTESIAN_POINT('Ctrl Pts',(18.7811102468205,-16.3910633800503,-14.7691219629677));
#54041=CARTESIAN_POINT('Ctrl Pts',(18.8650450584583,-16.3939774328894,-14.7732999727777));
#54042=CARTESIAN_POINT('Ctrl Pts',(18.9487268680229,-16.401021291318,-14.7774779825877));
#54043=CARTESIAN_POINT('Ctrl Pts',(19.032324781039,-16.4080580878126,-14.7816518036666));
#54044=CARTESIAN_POINT('Ctrl Pts',(19.1156697399224,-16.419216429775,-14.7858256247455));
#54045=CARTESIAN_POINT('Ctrl Pts',(19.1983256615619,-16.4344611859963,-14.7899994458244));
#54046=CARTESIAN_POINT('Ctrl Pts',(19.2809235142156,-16.4496952321861,-14.7941703346323));
#54047=CARTESIAN_POINT('Ctrl Pts',(19.3628328402599,-16.4690099061368,-14.7983412234403));
#54048=CARTESIAN_POINT('Ctrl Pts',(19.4436242958238,-16.4923184436239,-14.8025121122482));
#54049=CARTESIAN_POINT('Ctrl Pts',(19.5244040000537,-16.5156235908217,-14.8066823943892));
#54050=CARTESIAN_POINT('Ctrl Pts',(19.6040657115566,-16.5429213326382,-14.8108526765302));
#54051=CARTESIAN_POINT('Ctrl Pts',(19.6821928869636,-16.574074381081,-14.8150229586711));
#54052=CARTESIAN_POINT('Ctrl Pts',(19.7603101594137,-16.6052234807403,-14.8191927122109));
#54053=CARTESIAN_POINT('Ctrl Pts',(19.836892857112,-16.6402267397378,-14.8233624657506));
#54054=CARTESIAN_POINT('Ctrl Pts',(19.9115437773171,-16.6788984509042,-14.8275322192903));
#54055=CARTESIAN_POINT('Ctrl Pts',(19.9862468140621,-16.7175971602077,-14.8317048838875));
#54056=CARTESIAN_POINT('Ctrl Pts',(20.0590149720314,-16.7599692220591,-14.8358775484848));
#54057=CARTESIAN_POINT('Ctrl Pts',(20.1294756726678,-16.8057829450421,-14.8400502130821));
#54058=CARTESIAN_POINT('Ctrl Pts',(20.1856890006227,-16.8423329908352,-14.8433791519279));
#54059=CARTESIAN_POINT('Ctrl Pts',(20.2404341046543,-16.8810726448914,-14.8467080907738));
#54060=CARTESIAN_POINT('Ctrl Pts',(20.2935358883611,-16.9218650751948,-14.8500370296196));
#54061=CARTESIAN_POINT('Ctrl Pts',(20.2909850430174,-16.9251769135511,-14.0501277865439));
#54062=CARTESIAN_POINT('Ctrl Pts',(20.6448529485284,-17.1976900198726,-14.072256704909));
#54063=CARTESIAN_POINT('Ctrl Pts',(21.4803859272375,-18.2487089187753,-14.1367775588346));
#54064=CARTESIAN_POINT('Ctrl Pts',(21.2244734545047,-20.6727073586304,-14.2436903483206));
#54065=CARTESIAN_POINT('Ctrl Pts',(18.6352034645934,-21.9774803067,-14.3708661550021));
#54066=CARTESIAN_POINT('Ctrl Pts',(16.5197423660721,-20.7321305462553,-14.478539335638));
#54067=CARTESIAN_POINT('Ctrl Pts',(16.1790023713152,-19.4133917175901,-14.5438205807135));
#54068=CARTESIAN_POINT('Ctrl Pts',(16.1781028623508,-18.9514411453429,-14.5667098902285));
#54069=CARTESIAN_POINT('Origin',(18.734,-18.952,1.76670989022851));
#54070=CARTESIAN_POINT('',(20.293535888361,-16.9218650751948,-13.2501880128791));
#54071=CARTESIAN_POINT('',(20.293535888361,-16.9218650751948,-13.3166223775484));
#54072=CARTESIAN_POINT('',(20.293535888361,-16.9218650751948,1.76670989022851));
#54073=CARTESIAN_POINT('',(16.1740010575059,-18.949673107456,-13.8332901097715));
#54074=CARTESIAN_POINT('Ctrl Pts',(20.293535888361,-16.9218650751947,-13.3166223775484));
#54075=CARTESIAN_POINT('Ctrl Pts',(20.3602103318618,-16.9730839307523,-13.3207986507083));
#54076=CARTESIAN_POINT('Ctrl Pts',(20.4243042225914,-17.0275488083323,-13.3249749238681));
#54077=CARTESIAN_POINT('Ctrl Pts',(20.4855003242258,-17.0849577899156,-13.329151197028));
#54078=CARTESIAN_POINT('Ctrl Pts',(20.546804110082,-17.1424677916838,-13.3333348190011));
#54079=CARTESIAN_POINT('Ctrl Pts',(20.6051996004652,-17.2029319152096,-13.3375184409743));
#54080=CARTESIAN_POINT('Ctrl Pts',(20.6604076911347,-17.2660126312641,-13.3417020629474));
#54081=CARTESIAN_POINT('Ctrl Pts',(20.7059043008509,-17.3179970176855,-13.3451497571858));
#54082=CARTESIAN_POINT('Ctrl Pts',(20.7492369233109,-17.3717576847194,-13.3485974514241));
#54083=CARTESIAN_POINT('Ctrl Pts',(20.7902715950829,-17.4270911085396,-13.3520451456625));
#54084=CARTESIAN_POINT('Ctrl Pts',(20.8400773745207,-17.4942519796594,-13.3562297800555));
#54085=CARTESIAN_POINT('Ctrl Pts',(20.8866820202992,-17.5639804959204,-13.3604144144486));
#54086=CARTESIAN_POINT('Ctrl Pts',(20.9298102405872,-17.6359386840529,-13.3645990488416));
#54087=CARTESIAN_POINT('Ctrl Pts',(20.9728770731919,-17.7077944486113,-13.3687777269256));
#54088=CARTESIAN_POINT('Ctrl Pts',(21.0124770746365,-17.7818731899369,-13.3729564050095));
#54089=CARTESIAN_POINT('Ctrl Pts',(21.0483765860078,-17.8578057676359,-13.3771350830935));
#54090=CARTESIAN_POINT('Ctrl Pts',(21.0849195703199,-17.9350993822183,-13.3813886609789));
#54091=CARTESIAN_POINT('Ctrl Pts',(21.1176278099319,-18.0143135596366,-13.3856422388643));
#54092=CARTESIAN_POINT('Ctrl Pts',(21.1463023579538,-18.0950301441645,-13.3898958167498));
#54093=CARTESIAN_POINT('Ctrl Pts',(21.1744209939084,-18.1741818801958,-13.3940669307277));
#54094=CARTESIAN_POINT('Ctrl Pts',(21.1986607834443,-18.2547778355445,-13.3982380447057));
#54095=CARTESIAN_POINT('Ctrl Pts',(21.2188822787495,-18.3364026797032,-13.4024091586836));
#54096=CARTESIAN_POINT('Ctrl Pts',(21.2390969885367,-18.4180001338572,-13.406578873004));
#54097=CARTESIAN_POINT('Ctrl Pts',(21.2552959714612,-18.5006253449795,-13.4107485873244));
#54098=CARTESIAN_POINT('Ctrl Pts',(21.2673900009521,-18.5838490756821,-13.4149183016447));
#54099=CARTESIAN_POINT('Ctrl Pts',(21.2794836000854,-18.667069844927,-13.4190878675888));
#54100=CARTESIAN_POINT('Ctrl Pts',(21.2874724709,-18.750888636033,-13.4232574335328));
#54101=CARTESIAN_POINT('Ctrl Pts',(21.2913189573956,-18.83486866284,-13.4274269994769));
#54102=CARTESIAN_POINT('Ctrl Pts',(21.2953006816113,-18.9218013237892,-13.4317431622158));
#54103=CARTESIAN_POINT('Ctrl Pts',(21.2948432851383,-19.0089062426183,-13.4360593249547));
#54104=CARTESIAN_POINT('Ctrl Pts',(21.2899637772452,-19.0956981886119,-13.4403754876936));
#54105=CARTESIAN_POINT('Ctrl Pts',(21.2852432188086,-19.1796628960937,-13.4445510518853));
#54106=CARTESIAN_POINT('Ctrl Pts',(21.2763843217563,-19.26333424434,-13.448726616077));
#54107=CARTESIAN_POINT('Ctrl Pts',(21.2634552371752,-19.3462793465638,-13.4529021802687));
#54108=CARTESIAN_POINT('Ctrl Pts',(21.249873135268,-19.4334138087177,-13.4572886422812));
#54109=CARTESIAN_POINT('Ctrl Pts',(21.231798989378,-19.5197461599058,-13.4616751042938));
#54110=CARTESIAN_POINT('Ctrl Pts',(21.2093716504546,-19.6047903125243,-13.4660615663063));
#54111=CARTESIAN_POINT('Ctrl Pts',(21.1869443115312,-19.6898344651427,-13.4704480283188));
#54112=CARTESIAN_POINT('Ctrl Pts',(21.1601640287334,-19.7735898897036,-13.4748344903314));
#54113=CARTESIAN_POINT('Ctrl Pts',(21.1292278697972,-19.855594738667,-13.4792209523439));
#54114=CARTESIAN_POINT('Ctrl Pts',(21.099715129392,-19.9338264229693,-13.483405586737));
#54115=CARTESIAN_POINT('Ctrl Pts',(21.0663106928263,-20.0107562780701,-13.48759022113));
#54116=CARTESIAN_POINT('Ctrl Pts',(21.0291497318875,-20.0859698885847,-13.4917748555231));
#54117=CARTESIAN_POINT('Ctrl Pts',(20.9920416649769,-20.1610764418345,-13.495953533607));
#54118=CARTESIAN_POINT('Ctrl Pts',(20.9511878964455,-20.2344711938786,-13.500132211691));
#54119=CARTESIAN_POINT('Ctrl Pts',(20.9067723398086,-20.3057578658544,-13.5043108897749));
#54120=CARTESIAN_POINT('Ctrl Pts',(20.8615606662401,-20.3783223001923,-13.5085644676604));
#54121=CARTESIAN_POINT('Ctrl Pts',(20.8126584286878,-20.4487018853357,-13.5128180455458));
#54122=CARTESIAN_POINT('Ctrl Pts',(20.7603095437647,-20.5165029986702,-13.5170716234313));
#54123=CARTESIAN_POINT('Ctrl Pts',(20.7089755441263,-20.5829896551198,-13.5212427374092));
#54124=CARTESIAN_POINT('Ctrl Pts',(20.6543276385962,-20.6469965440968,-13.5254138513872));
#54125=CARTESIAN_POINT('Ctrl Pts',(20.596639573948,-20.7081816015329,-13.5295849653651));
#54126=CARTESIAN_POINT('Ctrl Pts',(20.5389708670871,-20.7693461277322,-13.5337546796855));
#54127=CARTESIAN_POINT('Ctrl Pts',(20.4782643424754,-20.8276903684964,-13.5379243940059));
#54128=CARTESIAN_POINT('Ctrl Pts',(20.4148326241775,-20.8829069603429,-13.5420941083262));
#54129=CARTESIAN_POINT('Ctrl Pts',(20.3514031630524,-20.938121587346,-13.5462636742703));
#54130=CARTESIAN_POINT('Ctrl Pts',(20.2852490485947,-20.9902084853113,-13.5504332402143));
#54131=CARTESIAN_POINT('Ctrl Pts',(20.216717166363,-21.0388995674379,-13.5546028061583));
#54132=CARTESIAN_POINT('Ctrl Pts',(20.1457757876953,-21.0893025679451,-13.5589189688973));
#54133=CARTESIAN_POINT('Ctrl Pts',(20.0722867555766,-21.1360662103826,-13.5632351316362));
#54134=CARTESIAN_POINT('Ctrl Pts',(19.9966672790439,-21.1789421506702,-13.5675512943751));
#54135=CARTESIAN_POINT('Ctrl Pts',(19.9235110990054,-21.2204214117129,-13.5717268585668));
#54136=CARTESIAN_POINT('Ctrl Pts',(19.848361583456,-21.2582621950959,-13.5759024227585));
#54137=CARTESIAN_POINT('Ctrl Pts',(19.7716196105685,-21.2922874916907,-13.5800779869502));
#54138=CARTESIAN_POINT('Ctrl Pts',(19.6910015830673,-21.3280313251289,-13.5844644489627));
#54139=CARTESIAN_POINT('Ctrl Pts',(19.6086265457421,-21.3595638930066,-13.5888509109752));
#54140=CARTESIAN_POINT('Ctrl Pts',(19.5249783787279,-21.3867388369977,-13.5932373729878));
#54141=CARTESIAN_POINT('Ctrl Pts',(19.4413302117137,-21.4139137809889,-13.5976238350003));
#54142=CARTESIAN_POINT('Ctrl Pts',(19.3564094950911,-21.4367310239951,-13.6020102970128));
#54143=CARTESIAN_POINT('Ctrl Pts',(19.2707112385803,-21.4551062794819,-13.6063967590254));
#54144=CARTESIAN_POINT('Ctrl Pts',(19.1889560858866,-21.4726360622251,-13.6105813934184));
#54145=CARTESIAN_POINT('Ctrl Pts',(19.1061890642126,-21.486188888916,-13.6147660278115));
#54146=CARTESIAN_POINT('Ctrl Pts',(19.022831797239,-21.4956541024486,-13.6189506622045));
#54147=CARTESIAN_POINT('Ctrl Pts',(18.9395931790174,-21.5051058434214,-13.6231293402885));
#54148=CARTESIAN_POINT('Ctrl Pts',(18.8557664374668,-21.5104814765754,-13.6273080183724));
#54149=CARTESIAN_POINT('Ctrl Pts',(18.7717843292959,-21.5117211458398,-13.6314866964564));
#54150=CARTESIAN_POINT('Ctrl Pts',(18.686296902193,-21.5129830352849,-13.6357402743418));
#54151=CARTESIAN_POINT('Ctrl Pts',(18.6006489552154,-21.5099591270341,-13.6399938522272));
#54152=CARTESIAN_POINT('Ctrl Pts',(18.5153034901261,-21.5026414559026,-13.6442474301127));
#54153=CARTESIAN_POINT('Ctrl Pts',(18.4316126134154,-21.4954656521053,-13.6484185440906));
#54154=CARTESIAN_POINT('Ctrl Pts',(18.3482130743116,-21.4841611267896,-13.6525896580686));
#54155=CARTESIAN_POINT('Ctrl Pts',(18.2655406684996,-21.4687729048784,-13.6567607720465));
#54156=CARTESIAN_POINT('Ctrl Pts',(18.1828960042119,-21.4533898466338,-13.6609304863669));
#54157=CARTESIAN_POINT('Ctrl Pts',(18.1009784405235,-21.4339258973908,-13.6651002006873));
#54158=CARTESIAN_POINT('Ctrl Pts',(18.0202156389588,-21.4104775544904,-13.6692699150076));
#54159=CARTESIAN_POINT('Ctrl Pts',(17.9394557112809,-21.3870300459825,-13.6734394809517));
#54160=CARTESIAN_POINT('Ctrl Pts',(17.8598509055781,-21.3595985548015,-13.6776090468957));
#54161=CARTESIAN_POINT('Ctrl Pts',(17.7818144029982,-21.3283296465058,-13.6817786128398));
#54162=CARTESIAN_POINT('Ctrl Pts',(17.7010342332561,-21.2959613619688,-13.6860947755787));
#54163=CARTESIAN_POINT('Ctrl Pts',(17.621935191217,-21.2594809885572,-13.6904109383176));
#54164=CARTESIAN_POINT('Ctrl Pts',(17.5449519222894,-21.219104909106,-13.6947271010565));
#54165=CARTESIAN_POINT('Ctrl Pts',(17.4704763752499,-21.1800440761962,-13.6989026652482));
#54166=CARTESIAN_POINT('Ctrl Pts',(17.3979812574151,-21.1373377246259,-13.7030782294399));
#54167=CARTESIAN_POINT('Ctrl Pts',(17.3278323932016,-21.091227117814,-13.7072537936316));
#54168=CARTESIAN_POINT('Ctrl Pts',(17.2541404766197,-21.0427875738696,-13.7116402556441));
#54169=CARTESIAN_POINT('Ctrl Pts',(17.1830385318335,-20.9905911845411,-13.7160267176566));
#54170=CARTESIAN_POINT('Ctrl Pts',(17.1149115381732,-20.9349655954603,-13.7204131796692));
#54171=CARTESIAN_POINT('Ctrl Pts',(17.0467845445129,-20.8793400063795,-13.7247996416817));
#54172=CARTESIAN_POINT('Ctrl Pts',(16.9816328807925,-20.8202856635707,-13.7291861036943));
#54173=CARTESIAN_POINT('Ctrl Pts',(16.9197953580219,-20.7581731691688,-13.7335725657068));
#54174=CARTESIAN_POINT('Ctrl Pts',(16.8612222805613,-20.6993396360182,-13.7377274633762));
#54175=CARTESIAN_POINT('Ctrl Pts',(16.8053896617352,-20.6375286216453,-13.7418823610455));
#54176=CARTESIAN_POINT('Ctrl Pts',(16.7526212754374,-20.5730300274365,-13.7460372587149));
#54177=CARTESIAN_POINT('Ctrl Pts',(16.7002946208399,-20.5090713601742,-13.7501573751423));
#54178=CARTESIAN_POINT('Ctrl Pts',(16.6509814300939,-20.4424702805592,-13.7542774915697));
#54179=CARTESIAN_POINT('Ctrl Pts',(16.6049624110076,-20.3735480803186,-13.7583976079971));
#54180=CARTESIAN_POINT('Ctrl Pts',(16.5589874739682,-20.3046919012954,-13.7625137777266));
#54181=CARTESIAN_POINT('Ctrl Pts',(16.5163007099123,-20.2335194044224,-13.7666299474561));
#54182=CARTESIAN_POINT('Ctrl Pts',(16.4771421768208,-20.1603843618463,-13.7707461171856));
#54183=CARTESIAN_POINT('Ctrl Pts',(16.4380086398887,-20.0872960037358,-13.7748596594307));
#54184=CARTESIAN_POINT('Ctrl Pts',(16.4023990866291,-20.0122480031431,-13.7789732016757));
#54185=CARTESIAN_POINT('Ctrl Pts',(16.3705090605919,-19.9356211564092,-13.7830867439208));
#54186=CARTESIAN_POINT('Ctrl Pts',(16.3380758082443,-19.8576890200784,-13.7872703577417));
#54187=CARTESIAN_POINT('Ctrl Pts',(16.3094902338592,-19.7781241832446,-13.7914539715626));
#54188=CARTESIAN_POINT('Ctrl Pts',(16.2849076425233,-19.6973500013747,-13.7956375853835));
#54189=CARTESIAN_POINT('Ctrl Pts',(16.2607361379239,-19.6179265800639,-13.7997512379815));
#54190=CARTESIAN_POINT('Ctrl Pts',(16.2404348481341,-19.5373344318006,-13.8038648905795));
#54191=CARTESIAN_POINT('Ctrl Pts',(16.2241009663662,-19.455990913573,-13.8079785431774));
#54192=CARTESIAN_POINT('Ctrl Pts',(16.2073503971231,-19.3725722716413,-13.8121971376098));
#54193=CARTESIAN_POINT('Ctrl Pts',(16.1947725425284,-19.2883639128979,-13.8164157320421));
#54194=CARTESIAN_POINT('Ctrl Pts',(16.1864159534739,-19.2038243949375,-13.8206343264745));
#54195=CARTESIAN_POINT('Ctrl Pts',(16.1780593644194,-19.1192848769771,-13.8248529209068));
#54196=CARTESIAN_POINT('Ctrl Pts',(16.1739240322153,-19.0344147354448,-13.8290715153392));
#54197=CARTESIAN_POINT('Ctrl Pts',(16.1740010575059,-18.949673107456,-13.8332901097715));
#54198=CARTESIAN_POINT('Ctrl Pts',(16.1735504202813,-18.9496726978525,-13.8332901097715));
#54199=CARTESIAN_POINT('Ctrl Pts',(16.1718449019213,-18.765781352641,-13.8424428639771));
#54200=CARTESIAN_POINT('Ctrl Pts',(16.2739023737919,-17.7320561796712,-13.8939875537431));
#54201=CARTESIAN_POINT('Ctrl Pts',(17.6781137265109,-16.1150307104843,-13.9879241790696));
#54202=CARTESIAN_POINT('Ctrl Pts',(19.6033699086469,-16.3924605121711,-14.0732424035937));
#54203=CARTESIAN_POINT('Ctrl Pts',(20.287632224731,-16.9120027987701,-14.1161686925573));
#54204=CARTESIAN_POINT('Ctrl Pts',(20.2961055948522,-16.9185282149957,-14.1167030459603));
#54205=CARTESIAN_POINT('',(16.1740010826188,-18.9543543591274,-13.7667098774921));
#54206=CARTESIAN_POINT('Ctrl Pts',(16.1744182719781,-18.9543537193378,-13.7667098902285));
#54207=CARTESIAN_POINT('Ctrl Pts',(16.1802301241212,-18.3145386211268,-13.7985275695778));
#54208=CARTESIAN_POINT('Ctrl Pts',(16.7471749526305,-16.8130883553205,-13.8727371844876));
#54209=CARTESIAN_POINT('Ctrl Pts',(18.7905373395045,-16.1321011936949,-13.9672098165927));
#54210=CARTESIAN_POINT('Ctrl Pts',(19.9669551317519,-16.6756419987287,-14.0298647693485));
#54211=CARTESIAN_POINT('Ctrl Pts',(20.2909850430174,-16.9251769135511,-14.0501277865439));
#54212=CARTESIAN_POINT('Ctrl Pts',(20.293535888361,-16.9218650751948,-13.2501880128791));
#54213=CARTESIAN_POINT('Ctrl Pts',(20.362109517474,-16.9745428722663,-13.2544909999071));
#54214=CARTESIAN_POINT('Ctrl Pts',(20.4280925084506,-17.030761458256,-13.2587939869351));
#54215=CARTESIAN_POINT('Ctrl Pts',(20.4911037568818,-17.0902303075966,-13.2630969739631));
#54216=CARTESIAN_POINT('Ctrl Pts',(20.5521864303202,-17.1478790035749,-13.2672682601696));
#54217=CARTESIAN_POINT('Ctrl Pts',(20.6104762833583,-17.2085815368414,-13.2714395463762));
#54218=CARTESIAN_POINT('Ctrl Pts',(20.6656594876492,-17.2720322551385,-13.2756108325828));
#54219=CARTESIAN_POINT('Ctrl Pts',(20.7208228024687,-17.3354601041358,-13.2797806153486));
#54220=CARTESIAN_POINT('Ctrl Pts',(20.772881390616,-17.4016338242775,-13.2839503981144));
#54221=CARTESIAN_POINT('Ctrl Pts',(20.8215597182926,-17.4702124232663,-13.2881201808803));
#54222=CARTESIAN_POINT('Ctrl Pts',(20.8702351033456,-17.5387868766527,-13.2922897115811));
#54223=CARTESIAN_POINT('Ctrl Pts',(20.9155303683828,-17.6097655443968,-13.296459242282));
#54224=CARTESIAN_POINT('Ctrl Pts',(20.9572123841055,-17.6827771294371,-13.3006287729829));
#54225=CARTESIAN_POINT('Ctrl Pts',(20.9989043835118,-17.7558062022249,-13.3047993023705));
#54226=CARTESIAN_POINT('Ctrl Pts',(21.0369811882063,-17.8308687591357,-13.308969831758));
#54227=CARTESIAN_POINT('Ctrl Pts',(21.0712555052538,-17.907568717837,-13.3131403611456));
#54228=CARTESIAN_POINT('Ctrl Pts',(21.105568902902,-17.9843561321234,-13.3173156458954));
#54229=CARTESIAN_POINT('Ctrl Pts',(21.1360709750617,-18.0627842525363,-13.3214909306453));
#54230=CARTESIAN_POINT('Ctrl Pts',(21.1626227268541,-18.1424373707935,-13.3256662153951));
#54231=CARTESIAN_POINT('Ctrl Pts',(21.1891927341781,-18.2221452541761,-13.3298443708422));
#54232=CARTESIAN_POINT('Ctrl Pts',(21.2118068930584,-18.3030793690225,-13.3340225262894));
#54233=CARTESIAN_POINT('Ctrl Pts',(21.2303768173696,-18.3848115077863,-13.3382006817365));
#54234=CARTESIAN_POINT('Ctrl Pts',(21.248976043095,-18.4666726113865,-13.3423854298796));
#54235=CARTESIAN_POINT('Ctrl Pts',(21.2635182251543,-18.5493337992202,-13.3465701780226));
#54236=CARTESIAN_POINT('Ctrl Pts',(21.2739665901778,-18.6323600137957,-13.3507549261656));
#54237=CARTESIAN_POINT('Ctrl Pts',(21.2762176599804,-18.6502477698261,-13.3516565179606));
#54238=CARTESIAN_POINT('Ctrl Pts',(21.278278897623,-18.6681524664035,-13.3525581097556));
#54239=CARTESIAN_POINT('Ctrl Pts',(21.2801502518719,-18.6860697555883,-13.3534597015506));
#54240=CARTESIAN_POINT('Ctrl Pts',(21.2888359269133,-18.7692307880738,-13.3576443359436));
#54241=CARTESIAN_POINT('Ctrl Pts',(21.2934592377886,-18.852972557727,-13.3618289703367));
#54242=CARTESIAN_POINT('Ctrl Pts',(21.2939552539536,-18.9368640244712,-13.3660136047297));
#54243=CARTESIAN_POINT('Ctrl Pts',(21.294450564101,-19.0206360820962,-13.3701922828137));
#54244=CARTESIAN_POINT('Ctrl Pts',(21.2908302458307,-19.1045569574875,-13.3743709608976));
#54245=CARTESIAN_POINT('Ctrl Pts',(21.2830810689264,-19.1881899744725,-13.3785496389816));
#54246=CARTESIAN_POINT('Ctrl Pts',(21.2751929935952,-19.2733220531809,-13.382803216867));
#54247=CARTESIAN_POINT('Ctrl Pts',(21.2630265340501,-19.3581553727241,-13.3870567947524));
#54248=CARTESIAN_POINT('Ctrl Pts',(21.2466232879999,-19.4422287349806,-13.3913103726379));
#54249=CARTESIAN_POINT('Ctrl Pts',(21.2305380508826,-19.5246721710542,-13.3954814866158));
#54250=CARTESIAN_POINT('Ctrl Pts',(21.2103789301821,-19.6063843810837,-13.3996526005938));
#54251=CARTESIAN_POINT('Ctrl Pts',(21.1862373001536,-19.686936884185,-13.4038237145717));
#54252=CARTESIAN_POINT('Ctrl Pts',(21.1621037710821,-19.7674623571159,-13.4079934288921));
#54253=CARTESIAN_POINT('Ctrl Pts',(21.133990518692,-19.8468284556772,-13.4121631432125));
#54254=CARTESIAN_POINT('Ctrl Pts',(21.1020392245072,-19.9246202913754,-13.4163328575329));
#54255=CARTESIAN_POINT('Ctrl Pts',(21.0700890672866,-20.0024093589063,-13.4205024234769));
#54256=CARTESIAN_POINT('Ctrl Pts',(21.0343013153839,-20.0786238497405,-13.4246719894209));
#54257=CARTESIAN_POINT('Ctrl Pts',(20.9948658827286,-20.1528686274167,-13.428841555365));
#54258=CARTESIAN_POINT('Ctrl Pts',(20.9540439489101,-20.2297237598852,-13.4331577181039));
#54259=CARTESIAN_POINT('Ctrl Pts',(20.9093133043205,-20.3044676260572,-13.4374738808428));
#54260=CARTESIAN_POINT('Ctrl Pts',(20.8609355752996,-20.3766912151498,-13.4417900435817));
#54261=CARTESIAN_POINT('Ctrl Pts',(20.8141337457131,-20.4465621284243,-13.4459656077734));
#54262=CARTESIAN_POINT('Ctrl Pts',(20.7639191093594,-20.514074089366,-13.4501411719651));
#54263=CARTESIAN_POINT('Ctrl Pts',(20.71057067018,-20.5788891744014,-13.4543167361568));
#54264=CARTESIAN_POINT('Ctrl Pts',(20.6545277281615,-20.6469779152985,-13.4587031981693));
#54265=CARTESIAN_POINT('Ctrl Pts',(20.5950264806454,-20.7120897510531,-13.4630896601819));
#54266=CARTESIAN_POINT('Ctrl Pts',(20.5324338669328,-20.7738769514622,-13.4674761221944));
#54267=CARTESIAN_POINT('Ctrl Pts',(20.4698412532202,-20.8356641518712,-13.4718625842069));
#54268=CARTESIAN_POINT('Ctrl Pts',(20.4041577572906,-20.8941263879947,-13.4762490462195));
#54269=CARTESIAN_POINT('Ctrl Pts',(20.3357880909558,-20.9489664272771,-13.480635508232));
#54270=CARTESIAN_POINT('Ctrl Pts',(20.2705642143173,-21.0012831950598,-13.4848201426251));
#54271=CARTESIAN_POINT('Ctrl Pts',(20.2026531489501,-21.0504984994761,-13.4890047770181));
#54272=CARTESIAN_POINT('Ctrl Pts',(20.1323821856731,-21.0963244303958,-13.4931894114112));
#54273=CARTESIAN_POINT('Ctrl Pts',(20.0622112444146,-21.1420851337748,-13.4973680894951));
#54274=CARTESIAN_POINT('Ctrl Pts',(19.9896874593621,-21.1844657972013,-13.5015467675791));
#54275=CARTESIAN_POINT('Ctrl Pts',(19.9151708448061,-21.2232189316268,-13.505725445663));
#54276=CARTESIAN_POINT('Ctrl Pts',(19.8393185734882,-21.2626666881356,-13.5099790235484));
#54277=CARTESIAN_POINT('Ctrl Pts',(19.7614017031197,-21.2983552879197,-13.5142326014339));
#54278=CARTESIAN_POINT('Ctrl Pts',(19.6818305443852,-21.3300700702735,-13.5184861793193));
#54279=CARTESIAN_POINT('Ctrl Pts',(19.603802027833,-21.361169999685,-13.5226572932973));
#54280=CARTESIAN_POINT('Ctrl Pts',(19.5241832407486,-21.3884486389203,-13.5268284072752));
#54281=CARTESIAN_POINT('Ctrl Pts',(19.4433839268982,-21.4117508906917,-13.5309995212532));
#54282=CARTESIAN_POINT('Ctrl Pts',(19.3626117260378,-21.4350453231675,-13.5351692355735));
#54283=CARTESIAN_POINT('Ctrl Pts',(19.2806602267964,-21.4543658907802,-13.5393389498939));
#54284=CARTESIAN_POINT('Ctrl Pts',(19.1979549742611,-21.4696071539973,-13.5435086642143));
#54285=CARTESIAN_POINT('Ctrl Pts',(19.1152526647336,-21.4848478748648,-13.5476782301583));
#54286=CARTESIAN_POINT('Ctrl Pts',(19.0317971078102,-21.4960094974156,-13.5518477961024));
#54287=CARTESIAN_POINT('Ctrl Pts',(18.9480233475311,-21.5030378293376,-13.5560173620464));
#54288=CARTESIAN_POINT('Ctrl Pts',(18.8613042051868,-21.5103132687396,-13.5603335247854));
#54289=CARTESIAN_POINT('Ctrl Pts',(18.7742445926768,-21.5131593125471,-13.5646496875243));
#54290=CARTESIAN_POINT('Ctrl Pts',(18.6873300367179,-21.5115745573293,-13.5689658502632));
#54291=CARTESIAN_POINT('Ctrl Pts',(18.6032467132776,-21.5100414253459,-13.5731414144549));
#54292=CARTESIAN_POINT('Ctrl Pts',(18.5192996078627,-21.5043618068031,-13.5773169786466));
#54293=CARTESIAN_POINT('Ctrl Pts',(18.4359238802629,-21.4945873882411,-13.5814925428382));
#54294=CARTESIAN_POINT('Ctrl Pts',(18.3483370428691,-21.4843192870339,-13.5858790048508));
#54295=CARTESIAN_POINT('Ctrl Pts',(18.2613813964208,-21.4695319558998,-13.5902654668633));
#54296=CARTESIAN_POINT('Ctrl Pts',(18.1755479442734,-21.4503457129578,-13.5946519288759));
#54297=CARTESIAN_POINT('Ctrl Pts',(18.089714492126,-21.4311594700159,-13.5990383908884));
#54298=CARTESIAN_POINT('Ctrl Pts',(18.0050037728348,-21.4075745441673,-13.6034248529009));
#54299=CARTESIAN_POINT('Ctrl Pts',(17.921884774769,-21.379770347654,-13.6078113149135));
#54300=CARTESIAN_POINT('Ctrl Pts',(17.842590205016,-21.353245463438,-13.6119959493065));
#54301=CARTESIAN_POINT('Ctrl Pts',(17.7644489508446,-21.3227823154618,-13.6161805836996));
#54302=CARTESIAN_POINT('Ctrl Pts',(17.6878802554244,-21.2885002632162,-13.6203652180926));
#54303=CARTESIAN_POINT('Ctrl Pts',(17.6114205460648,-21.2542670072286,-13.6245438961766));
#54304=CARTESIAN_POINT('Ctrl Pts',(17.536529365682,-21.2162258304372,-13.6287225742605));
#54305=CARTESIAN_POINT('Ctrl Pts',(17.4636096823068,-21.1745454867587,-13.6329012523445));
#54306=CARTESIAN_POINT('Ctrl Pts',(17.3893829660135,-21.1321180528749,-13.6371548302299));
#54307=CARTESIAN_POINT('Ctrl Pts',(17.3171995773182,-21.0859198576823,-13.6414084081153));
#54308=CARTESIAN_POINT('Ctrl Pts',(17.2474621052952,-21.0361797157651,-13.6456619860008));
#54309=CARTESIAN_POINT('Ctrl Pts',(17.1790766302489,-20.9874038835589,-13.6498330999787));
#54310=CARTESIAN_POINT('Ctrl Pts',(17.1130434722312,-20.9352224936048,-13.6540042139567));
#54311=CARTESIAN_POINT('Ctrl Pts',(17.0497148300457,-20.879896124347,-13.6581753279346));
#54312=CARTESIAN_POINT('Ctrl Pts',(16.9864074383977,-20.8245883203866,-13.662345042255));
#54313=CARTESIAN_POINT('Ctrl Pts',(16.9258031063752,-20.7661379354358,-13.6665147565754));
#54314=CARTESIAN_POINT('Ctrl Pts',(16.8682208314237,-20.7048457131495,-13.6706844708957));
#54315=CARTESIAN_POINT('Ctrl Pts',(16.8106406054966,-20.6435556719036,-13.6748540368398));
#54316=CARTESIAN_POINT('Ctrl Pts',(16.7560825371937,-20.5794243302491,-13.6790236027838));
#54317=CARTESIAN_POINT('Ctrl Pts',(16.7048276747609,-20.512788158106,-13.6831931687279));
#54318=CARTESIAN_POINT('Ctrl Pts',(16.6517707545947,-20.4438091403549,-13.6875093314668));
#54319=CARTESIAN_POINT('Ctrl Pts',(16.6022539651132,-20.3721462932498,-13.6918254942057));
#54320=CARTESIAN_POINT('Ctrl Pts',(16.5565412927829,-20.2982071082729,-13.6961416569446));
#54321=CARTESIAN_POINT('Ctrl Pts',(16.5123177059456,-20.2266764844696,-13.7003172211363));
#54322=CARTESIAN_POINT('Ctrl Pts',(16.4716543903427,-20.1530159839383,-13.704492785328));
#54323=CARTESIAN_POINT('Ctrl Pts',(16.4347434295141,-20.0776194841408,-13.7086683495197));
#54324=CARTESIAN_POINT('Ctrl Pts',(16.3959681838015,-19.9984148863766,-13.7130548115322));
#54325=CARTESIAN_POINT('Ctrl Pts',(16.3613345469612,-19.9172948468639,-13.7174412735447));
#54326=CARTESIAN_POINT('Ctrl Pts',(16.3310071212994,-19.8347373476376,-13.7218277355573));
#54327=CARTESIAN_POINT('Ctrl Pts',(16.3006796956376,-19.7521798484113,-13.7262141975698));
#54328=CARTESIAN_POINT('Ctrl Pts',(16.2746585801944,-19.668185466211,-13.7306006595824));
#54329=CARTESIAN_POINT('Ctrl Pts',(16.253046772176,-19.5832456584798,-13.7349871215949));
#54330=CARTESIAN_POINT('Ctrl Pts',(16.2263033450823,-19.4781373050522,-13.7404151277539));
#54331=CARTESIAN_POINT('Ctrl Pts',(16.2062281520528,-19.3712684537335,-13.745843133913));
#54332=CARTESIAN_POINT('Ctrl Pts',(16.193006541868,-19.2633715557504,-13.751271140072));
#54333=CARTESIAN_POINT('Ctrl Pts',(16.1804712473274,-19.161075437704,-13.7564173858787));
#54334=CARTESIAN_POINT('Ctrl Pts',(16.1740962693079,-19.0578550605845,-13.7615636316854));
#54335=CARTESIAN_POINT('Ctrl Pts',(16.1740010826188,-18.9543543591274,-13.7667098774921));
#54336=CARTESIAN_POINT('Origin',(18.734,-18.952,1.76670989022851));
#54337=CARTESIAN_POINT('',(20.2954167197789,-16.919379410122,-12.4500366865268));
#54338=CARTESIAN_POINT('',(20.293535888361,-16.9218650751948,-12.5167193514887));
#54339=CARTESIAN_POINT('',(20.293535888361,-16.9218650751948,1.76670989022851));
#54340=CARTESIAN_POINT('',(16.174000001606,-18.9520906788002,-13.0332901097364));
#54341=CARTESIAN_POINT('Ctrl Pts',(20.293535888361,-16.9218650751948,-12.5167193514888));
#54342=CARTESIAN_POINT('Ctrl Pts',(20.3602126490049,-16.9730857107659,-12.5208888673399));
#54343=CARTESIAN_POINT('Ctrl Pts',(20.4243799356247,-17.0276073698207,-12.5250583831911));
#54344=CARTESIAN_POINT('Ctrl Pts',(20.4857025055872,-17.085147479869,-12.5292278990423));
#54345=CARTESIAN_POINT('Ctrl Pts',(20.5470295704357,-17.1426918075526,-12.533397720515));
#54346=CARTESIAN_POINT('Ctrl Pts',(20.6055111700133,-17.2032547098065,-12.5375675419877));
#54347=CARTESIAN_POINT('Ctrl Pts',(20.6608480451726,-17.2665159120257,-12.5417373634604));
#54348=CARTESIAN_POINT('Ctrl Pts',(20.7162427485479,-17.3298432235519,-12.5459115424856));
#54349=CARTESIAN_POINT('Ctrl Pts',(20.768485861661,-17.3958741188096,-12.5500857215108));
#54350=CARTESIAN_POINT('Ctrl Pts',(20.8173179976359,-17.4642546855304,-12.554259900536));
#54351=CARTESIAN_POINT('Ctrl Pts',(20.866176429233,-17.5326720745099,-12.5584363273153));
#54352=CARTESIAN_POINT('Ctrl Pts',(20.9116199773849,-17.6034412672135,-12.5626127540945));
#54353=CARTESIAN_POINT('Ctrl Pts',(20.9534335859414,-17.6761808288023,-12.5667891808738));
#54354=CARTESIAN_POINT('Ctrl Pts',(20.9953200425185,-17.7490471178675,-12.570972883859));
#54355=CARTESIAN_POINT('Ctrl Pts',(21.033563718021,-17.8238902224893,-12.5751565868442));
#54356=CARTESIAN_POINT('Ctrl Pts',(21.0679964529279,-17.9003058630381,-12.5793402898293));
#54357=CARTESIAN_POINT('Ctrl Pts',(21.0944703234963,-17.9590586104676,-12.5825569617442));
#54358=CARTESIAN_POINT('Ctrl Pts',(21.1186923494888,-18.0187404702052,-12.585773633659));
#54359=CARTESIAN_POINT('Ctrl Pts',(21.1406062076889,-18.0791617783844,-12.5889903055739));
#54360=CARTESIAN_POINT('Ctrl Pts',(21.1691143947643,-18.1577650960285,-12.5931749399669));
#54361=CARTESIAN_POINT('Ctrl Pts',(21.193820633909,-18.2379128391996,-12.59735957436));
#54362=CARTESIAN_POINT('Ctrl Pts',(21.2145578396958,-18.319202398927,-12.601544208753));
#54363=CARTESIAN_POINT('Ctrl Pts',(21.2352655286369,-18.4003762530279,-12.605722886837));
#54364=CARTESIAN_POINT('Ctrl Pts',(21.25201529302,-18.4826882535134,-12.6099015649209));
#54365=CARTESIAN_POINT('Ctrl Pts',(21.2646888572063,-18.5657178388643,-12.6140802430049));
#54366=CARTESIAN_POINT('Ctrl Pts',(21.2775895859224,-18.6502356698601,-12.6183338208903));
#54367=CARTESIAN_POINT('Ctrl Pts',(21.2862663809329,-18.735496610923,-12.6225873987757));
#54368=CARTESIAN_POINT('Ctrl Pts',(21.2906482513971,-18.8210430657493,-12.6268409766612));
#54369=CARTESIAN_POINT('Ctrl Pts',(21.2949451707518,-18.9049310356185,-12.6310120906391));
#54370=CARTESIAN_POINT('Ctrl Pts',(21.2951121858363,-18.9890930669704,-12.6351832046171));
#54371=CARTESIAN_POINT('Ctrl Pts',(21.2911345092731,-19.073091294008,-12.639354318595));
#54372=CARTESIAN_POINT('Ctrl Pts',(21.2871581674578,-19.1570613346294,-12.6435240329154));
#54373=CARTESIAN_POINT('Ctrl Pts',(21.2790399178704,-19.2408672209645,-12.6476937472358));
#54374=CARTESIAN_POINT('Ctrl Pts',(21.2668170738604,-19.3240721305894,-12.6518634615562));
#54375=CARTESIAN_POINT('Ctrl Pts',(21.2545946647916,-19.4072740794265,-12.6560330275002));
#54376=CARTESIAN_POINT('Ctrl Pts',(21.2382680194079,-19.4898746390487,-12.6602025934442));
#54377=CARTESIAN_POINT('Ctrl Pts',(21.2179260255778,-19.5714445087795,-12.6643721593883));
#54378=CARTESIAN_POINT('Ctrl Pts',(21.1968688323393,-19.6558822745029,-12.6686883221272));
#54379=CARTESIAN_POINT('Ctrl Pts',(21.1715088054102,-19.7392150119469,-12.6730044848661));
#54380=CARTESIAN_POINT('Ctrl Pts',(21.1420010732758,-19.8209826414278,-12.6773206476051));
#54381=CARTESIAN_POINT('Ctrl Pts',(21.113454552412,-19.9000866989788,-12.6814962117967));
#54382=CARTESIAN_POINT('Ctrl Pts',(21.0810266246877,-19.9777256330122,-12.6856717759884));
#54383=CARTESIAN_POINT('Ctrl Pts',(21.0449064462655,-20.0535041518799,-12.6898473401801));
#54384=CARTESIAN_POINT('Ctrl Pts',(21.0069619234988,-20.1331100635892,-12.6942338021926));
#54385=CARTESIAN_POINT('Ctrl Pts',(20.9649426346355,-20.2106621684913,-12.6986202642052));
#54386=CARTESIAN_POINT('Ctrl Pts',(20.9191207015645,-20.2857344261862,-12.7030067262177));
#54387=CARTESIAN_POINT('Ctrl Pts',(20.8732987684935,-20.3608066838811,-12.7073931882303));
#54388=CARTESIAN_POINT('Ctrl Pts',(20.8236745814507,-20.433398658303,-12.7117796502428));
#54389=CARTESIAN_POINT('Ctrl Pts',(20.7705691100602,-20.5031241923033,-12.7161661122553));
#54390=CARTESIAN_POINT('Ctrl Pts',(20.7199071001297,-20.5696415511261,-12.7203507466484));
#54391=CARTESIAN_POINT('Ctrl Pts',(20.6658885504363,-20.6337980416559,-12.7245353810414));
#54392=CARTESIAN_POINT('Ctrl Pts',(20.6087615512374,-20.6952352468906,-12.7287200154345));
#54393=CARTESIAN_POINT('Ctrl Pts',(20.5517158652512,-20.7565850038679,-12.7328986935184));
#54394=CARTESIAN_POINT('Ctrl Pts',(20.4915708287757,-20.8152228296984,-12.7370773716023));
#54395=CARTESIAN_POINT('Ctrl Pts',(20.4286160471336,-20.8708216313137,-12.7412560496863));
#54396=CARTESIAN_POINT('Ctrl Pts',(20.3645328462752,-20.9274170014899,-12.7455096275717));
#54397=CARTESIAN_POINT('Ctrl Pts',(20.2975384722485,-20.9808629432569,-12.7497632054571));
#54398=CARTESIAN_POINT('Ctrl Pts',(20.2279792651332,-21.0308520763518,-12.7540167833426));
#54399=CARTESIAN_POINT('Ctrl Pts',(20.1597685989815,-21.0798720725558,-12.7581878973205));
#54400=CARTESIAN_POINT('Ctrl Pts',(20.0890920516424,-21.1255678171228,-12.7623590112985));
#54401=CARTESIAN_POINT('Ctrl Pts',(20.0163097948304,-21.1676898677572,-12.7665301252764));
#54402=CARTESIAN_POINT('Ctrl Pts',(19.9435519608075,-21.2097977839308,-12.7706998395968));
#54403=CARTESIAN_POINT('Ctrl Pts',(19.8686902184419,-21.2483341575376,-12.7748695539171));
#54404=CARTESIAN_POINT('Ctrl Pts',(19.7921120632718,-21.2830939195062,-12.7790392682375));
#54405=CARTESIAN_POINT('Ctrl Pts',(19.715536633081,-21.3178524445734,-12.7832088341816));
#54406=CARTESIAN_POINT('Ctrl Pts',(19.6372453307739,-21.3488344358332,-12.7873784001256));
#54407=CARTESIAN_POINT('Ctrl Pts',(19.5576472435982,-21.3758822616029,-12.7915479660696));
#54408=CARTESIAN_POINT('Ctrl Pts',(19.4752505858723,-21.4038810555595,-12.7958641288086));
#54409=CARTESIAN_POINT('Ctrl Pts',(19.3914540397878,-21.4276637164715,-12.8001802915475));
#54410=CARTESIAN_POINT('Ctrl Pts',(19.3067284276564,-21.4471116504386,-12.8044964542864));
#54411=CARTESIAN_POINT('Ctrl Pts',(19.2247627434287,-21.4659260700022,-12.8086720184781));
#54412=CARTESIAN_POINT('Ctrl Pts',(19.1419280643015,-21.4806837970704,-12.8128475826698));
#54413=CARTESIAN_POINT('Ctrl Pts',(19.058659154638,-21.4913299181693,-12.8170231468614));
#54414=CARTESIAN_POINT('Ctrl Pts',(18.9711845303003,-21.5025137495362,-12.821409608874));
#54415=CARTESIAN_POINT('Ctrl Pts',(18.8832312388616,-21.5091596607904,-12.8257960708865));
#54416=CARTESIAN_POINT('Ctrl Pts',(18.7953048072929,-21.5112658557881,-12.830182532899));
#54417=CARTESIAN_POINT('Ctrl Pts',(18.7073783757242,-21.5133720507858,-12.8345689949116));
#54418=CARTESIAN_POINT('Ctrl Pts',(18.6194793819154,-21.5109386216197,-12.8389554569241));
#54419=CARTESIAN_POINT('Ctrl Pts',(18.5321062576875,-21.5040264334084,-12.8433419189367));
#54420=CARTESIAN_POINT('Ctrl Pts',(18.4487533004234,-21.497432285223,-12.8475265533297));
#54421=CARTESIAN_POINT('Ctrl Pts',(18.3655686284663,-21.4867379250515,-12.8517111877228));
#54422=CARTESIAN_POINT('Ctrl Pts',(18.2829879003454,-21.4719579532137,-12.8558958221158));
#54423=CARTESIAN_POINT('Ctrl Pts',(18.2005247156697,-21.4571990188365,-12.8600745001997));
#54424=CARTESIAN_POINT('Ctrl Pts',(18.1186642162802,-21.4383661042868,-12.8642531782836));
#54425=CARTESIAN_POINT('Ctrl Pts',(18.0378381935519,-21.4155256725358,-12.8684318563676));
#54426=CARTESIAN_POINT('Ctrl Pts',(17.9555634224545,-21.3922758424606,-12.872685434253));
#54427=CARTESIAN_POINT('Ctrl Pts',(17.8743610594202,-21.3648734505898,-12.8769390121385));
#54428=CARTESIAN_POINT('Ctrl Pts',(17.7946770299223,-21.3334433350144,-12.8811925900239));
#54429=CARTESIAN_POINT('Ctrl Pts',(17.7165378308269,-21.3026225535603,-12.8853637040018));
#54430=CARTESIAN_POINT('Ctrl Pts',(17.6398590665666,-21.2679290019,-12.8895348179798));
#54431=CARTESIAN_POINT('Ctrl Pts',(17.5650454327544,-21.2295305090636,-12.8937059319577));
#54432=CARTESIAN_POINT('Ctrl Pts',(17.4902569033794,-21.1911449012123,-12.8978756462781));
#54433=CARTESIAN_POINT('Ctrl Pts',(17.4173326704122,-21.1490570311436,-12.9020453605985));
#54434=CARTESIAN_POINT('Ctrl Pts',(17.3466549084742,-21.103481721284,-12.9062150749189));
#54435=CARTESIAN_POINT('Ctrl Pts',(17.2759796615541,-21.0579080331895,-12.9103846408629));
#54436=CARTESIAN_POINT('Ctrl Pts',(17.207551112884,-21.0088474020654,-12.9145542068069));
#54437=CARTESIAN_POINT('Ctrl Pts',(17.1417232369319,-20.9565584825076,-12.918723772751));
#54438=CARTESIAN_POINT('Ctrl Pts',(17.0735809340686,-20.9024311490435,-12.9230399354899));
#54439=CARTESIAN_POINT('Ctrl Pts',(17.0082259988608,-20.8448446181551,-12.9273560982288));
#54440=CARTESIAN_POINT('Ctrl Pts',(16.9460129971982,-20.7841305842685,-12.9316722609678));
#54441=CARTESIAN_POINT('Ctrl Pts',(16.8858265775212,-20.7253943036498,-12.9358478251595));
#54442=CARTESIAN_POINT('Ctrl Pts',(16.8285808237902,-20.6637315251356,-12.9400233893511));
#54443=CARTESIAN_POINT('Ctrl Pts',(16.7745572392501,-20.5994780931304,-12.9441989535428));
#54444=CARTESIAN_POINT('Ctrl Pts',(16.7178050518835,-20.5319793730225,-12.9485854155554));
#54445=CARTESIAN_POINT('Ctrl Pts',(16.6646094437671,-20.4616218795447,-12.9529718775679));
#54446=CARTESIAN_POINT('Ctrl Pts',(16.6152455573351,-20.3888297086599,-12.9573583395805));
#54447=CARTESIAN_POINT('Ctrl Pts',(16.565881670903,-20.316037537775,-12.961744801593));
#54448=CARTESIAN_POINT('Ctrl Pts',(16.5203497415207,-20.240811225245,-12.9661312636056));
#54449=CARTESIAN_POINT('Ctrl Pts',(16.4788683829465,-20.1636028184871,-12.9705177256181));
#54450=CARTESIAN_POINT('Ctrl Pts',(16.4371381237558,-20.0859311380873,-12.9749305077209));
#54451=CARTESIAN_POINT('Ctrl Pts',(16.3993648293879,-20.0059905501582,-12.9793432898236));
#54452=CARTESIAN_POINT('Ctrl Pts',(16.3657873879881,-19.9241980375972,-12.9837560719264));
#54453=CARTESIAN_POINT('Ctrl Pts',(16.3323070847553,-19.8426421474352,-12.9881560880307));
#54454=CARTESIAN_POINT('Ctrl Pts',(16.302998596953,-19.7592453620159,-12.9925561041351));
#54455=CARTESIAN_POINT('Ctrl Pts',(16.278054237255,-19.6744475139794,-12.9969561202394));
#54456=CARTESIAN_POINT('Ctrl Pts',(16.2531532512186,-19.5897971138313,-13.0013484855236));
#54457=CARTESIAN_POINT('Ctrl Pts',(16.2326014031163,-19.5037508664346,-13.0057408508078));
#54458=CARTESIAN_POINT('Ctrl Pts',(16.2165427462274,-19.4167676574675,-13.010133216092));
#54459=CARTESIAN_POINT('Ctrl Pts',(16.200521001668,-19.3299843875664,-13.0145154851125));
#54460=CARTESIAN_POINT('Ctrl Pts',(16.1889719431305,-19.2422688247292,-13.018897754133));
#54461=CARTESIAN_POINT('Ctrl Pts',(16.1819893075699,-19.1540926166946,-13.0232800231536));
#54462=CARTESIAN_POINT('Ctrl Pts',(16.176672671659,-19.0869545296414,-13.0266167186812));
#54463=CARTESIAN_POINT('Ctrl Pts',(16.1740023911013,-19.0195497546633,-13.0299534142088));
#54464=CARTESIAN_POINT('Ctrl Pts',(16.174000001606,-18.9520906788001,-13.0332901097364));
#54465=CARTESIAN_POINT('Ctrl Pts',(16.174000001606,-18.9520906780897,-13.0332901097715));
#54466=CARTESIAN_POINT('Ctrl Pts',(16.1739968821085,-18.8640218456489,-13.0376462156856));
#54467=CARTESIAN_POINT('Ctrl Pts',(16.1785426714359,-18.776035607655,-13.0420023215996));
#54468=CARTESIAN_POINT('Ctrl Pts',(16.1875860737584,-18.6886065372053,-13.0463584275137));
#54469=CARTESIAN_POINT('Ctrl Pts',(16.1966529338892,-18.6009506832622,-13.050725832792));
#54470=CARTESIAN_POINT('Ctrl Pts',(16.2102406836425,-18.5138552818865,-13.0550932380704));
#54471=CARTESIAN_POINT('Ctrl Pts',(16.2282463851318,-18.4277874271108,-13.0594606433487));
#54472=CARTESIAN_POINT('Ctrl Pts',(16.2462755658188,-18.3416073409855,-13.0638337436661));
#54473=CARTESIAN_POINT('Ctrl Pts',(16.2687340840993,-18.2564578570398,-13.0682068439834));
#54474=CARTESIAN_POINT('Ctrl Pts',(16.2954690366781,-18.1727909517206,-13.0725799443007));
#54475=CARTESIAN_POINT('Ctrl Pts',(16.3222767415772,-18.0888963683653,-13.0769649448896));
#54476=CARTESIAN_POINT('Ctrl Pts',(16.3533840099471,-18.0064928038111,-13.0813499454785));
#54477=CARTESIAN_POINT('Ctrl Pts',(16.3885892814888,-17.9260133716794,-13.0857349460673));
#54478=CARTESIAN_POINT('Ctrl Pts',(16.4205927188907,-17.8528533488879,-13.0897211414781));
#54479=CARTESIAN_POINT('Ctrl Pts',(16.4559819492917,-17.7812832866316,-13.0937073368888));
#54480=CARTESIAN_POINT('Ctrl Pts',(16.4945737975983,-17.7116088181558,-13.0976935322996));
#54481=CARTESIAN_POINT('Ctrl Pts',(16.5350868078939,-17.638465846711,-13.1018781666926));
#54482=CARTESIAN_POINT('Ctrl Pts',(16.5792624158945,-17.5671736686978,-13.1060628010856));
#54483=CARTESIAN_POINT('Ctrl Pts',(16.6269069559,-17.4981228031552,-13.1102474354787));
#54484=CARTESIAN_POINT('Ctrl Pts',(16.6744836797999,-17.4291702229729,-13.1144261135626));
#54485=CARTESIAN_POINT('Ctrl Pts',(16.7255192690589,-17.3624529938655,-13.1186047916466));
#54486=CARTESIAN_POINT('Ctrl Pts',(16.779774450421,-17.2983366420662,-13.1227834697305));
#54487=CARTESIAN_POINT('Ctrl Pts',(16.8350021169166,-17.2330710507404,-13.1270370476159));
#54488=CARTESIAN_POINT('Ctrl Pts',(16.8935656995715,-17.1705009170566,-13.1312906255014));
#54489=CARTESIAN_POINT('Ctrl Pts',(16.9551669364595,-17.110980463967,-13.1355442033868));
#54490=CARTESIAN_POINT('Ctrl Pts',(17.0155739131654,-17.0526139310053,-13.1397153173648));
#54491=CARTESIAN_POINT('Ctrl Pts',(17.0789014673906,-16.9971802202222,-13.1438864313427));
#54492=CARTESIAN_POINT('Ctrl Pts',(17.1448292745174,-16.9449782250137,-13.1480575453207));
#54493=CARTESIAN_POINT('Ctrl Pts',(17.2107349589319,-16.8927937466888,-13.152227259641));
#54494=CARTESIAN_POINT('Ctrl Pts',(17.2792388030076,-16.8438391155734,-13.1563969739614));
#54495=CARTESIAN_POINT('Ctrl Pts',(17.3499870301182,-16.7983732683683,-13.1605666882818));
#54496=CARTESIAN_POINT('Ctrl Pts',(17.4207327397034,-16.752909039033,-13.1647362542258));
#54497=CARTESIAN_POINT('Ctrl Pts',(17.4937222860638,-16.7109335947647,-13.1689058201699));
#54498=CARTESIAN_POINT('Ctrl Pts',(17.5685736694554,-16.6726620548779,-13.1730753861139));
#54499=CARTESIAN_POINT('Ctrl Pts',(17.6460567351476,-16.6330449348619,-13.1773915488529));
#54500=CARTESIAN_POINT('Ctrl Pts',(17.7255345286225,-16.5973972639687,-13.1817077115918));
#54501=CARTESIAN_POINT('Ctrl Pts',(17.8065583197874,-16.5659044592045,-13.1860238743307));
#54502=CARTESIAN_POINT('Ctrl Pts',(17.8849427694772,-16.535437529243,-13.1901994385224));
#54503=CARTESIAN_POINT('Ctrl Pts',(17.9647735800337,-16.5088590368059,-13.1943750027141));
#54504=CARTESIAN_POINT('Ctrl Pts',(18.0456284938944,-16.4862861744351,-13.1985505669058));
#54505=CARTESIAN_POINT('Ctrl Pts',(18.1305671972398,-16.4625732104478,-13.2029370289183));
#54506=CARTESIAN_POINT('Ctrl Pts',(18.2166356079047,-16.4432812873466,-13.2073234909308));
#54507=CARTESIAN_POINT('Ctrl Pts',(18.3033337697292,-16.4284852688949,-13.2117099529434));
#54508=CARTESIAN_POINT('Ctrl Pts',(18.3900319315538,-16.4136892504433,-13.2160964149559));
#54509=CARTESIAN_POINT('Ctrl Pts',(18.4773592594053,-16.4033891290646,-13.2204828769685));
#54510=CARTESIAN_POINT('Ctrl Pts',(18.5648137584887,-16.3975967398073,-13.224869338981));
#54511=CARTESIAN_POINT('Ctrl Pts',(18.6482240610121,-16.3920722105338,-13.2290529559168));
#54512=CARTESIAN_POINT('Ctrl Pts',(18.7320604262271,-16.3906271591048,-13.2332365728525));
#54513=CARTESIAN_POINT('Ctrl Pts',(18.8158899787624,-16.3933100947207,-13.2374201897883));
#54514=CARTESIAN_POINT('Ctrl Pts',(18.8996093084473,-16.3959895026926,-13.2415983059171));
#54515=CARTESIAN_POINT('Ctrl Pts',(18.9833213878534,-16.4027861079022,-13.245776422046));
#54516=CARTESIAN_POINT('Ctrl Pts',(19.0665895300201,-16.4136965893493,-13.2499545381748));
#54517=CARTESIAN_POINT('Ctrl Pts',(19.1497731758387,-16.4245959993852,-13.2541284145602));
#54518=CARTESIAN_POINT('Ctrl Pts',(19.2325133255144,-16.4396009359381,-13.2583022909457));
#54519=CARTESIAN_POINT('Ctrl Pts',(19.3143759725404,-16.4586561146729,-13.2624761673311));
#54520=CARTESIAN_POINT('Ctrl Pts',(19.396180111325,-16.4776976744371,-13.2666470605958));
#54521=CARTESIAN_POINT('Ctrl Pts',(19.4771075468216,-16.5007836209281,-13.2708179538604));
#54522=CARTESIAN_POINT('Ctrl Pts',(19.5567334109211,-16.5278074056391,-13.274988847125));
#54523=CARTESIAN_POINT('Ctrl Pts',(19.6363403165266,-16.554824756131,-13.2791587473222));
#54524=CARTESIAN_POINT('Ctrl Pts',(19.7146458288506,-16.5857779414159,-13.2833286475194));
#54525=CARTESIAN_POINT('Ctrl Pts',(19.7912403187458,-16.6205105815341,-13.2874985477165));
#54526=CARTESIAN_POINT('Ctrl Pts',(19.8678247271481,-16.655238650085,-13.2916678990646));
#54527=CARTESIAN_POINT('Ctrl Pts',(19.9426981444006,-16.6937449890619,-13.2958372504126));
#54528=CARTESIAN_POINT('Ctrl Pts',(20.0154725000699,-16.7358257668756,-13.3000066017606));
#54529=CARTESIAN_POINT('Ctrl Pts',(20.0882810786158,-16.7779263336005,-13.3041779137883));
#54530=CARTESIAN_POINT('Ctrl Pts',(20.1589882301708,-16.8236044584369,-13.308349225816));
#54531=CARTESIAN_POINT('Ctrl Pts',(20.2272328428162,-16.8726117060214,-13.3125205378436));
#54532=CARTESIAN_POINT('Ctrl Pts',(20.2496021804837,-16.8886753867558,-13.3138878177452));
#54533=CARTESIAN_POINT('Ctrl Pts',(20.2717071853379,-16.905096413494,-13.3152550976468));
#54534=CARTESIAN_POINT('Ctrl Pts',(20.293535888361,-16.9218650751947,-13.3166223775484));
#54535=CARTESIAN_POINT('',(16.1736697275687,-18.9513574892655,-12.9667098340851));
#54536=CARTESIAN_POINT('Ctrl Pts',(16.1740000808904,-18.9513564484225,-12.9667098902285));
#54537=CARTESIAN_POINT('Ctrl Pts',(16.1740088273484,-18.9165636940743,-12.9684506873211));
#54538=CARTESIAN_POINT('Ctrl Pts',(16.1747268399112,-18.881780730387,-12.9701914844137));
#54539=CARTESIAN_POINT('Ctrl Pts',(16.1761531171477,-18.8470270326105,-12.9719322815063));
#54540=CARTESIAN_POINT('Ctrl Pts',(16.1795816894971,-18.7634839708603,-12.9761169158993));
#54541=CARTESIAN_POINT('Ctrl Pts',(16.1871139062631,-18.6799535889704,-12.9803015502924));
#54542=CARTESIAN_POINT('Ctrl Pts',(16.1987516982625,-18.5968717857769,-12.9844861846854));
#54543=CARTESIAN_POINT('Ctrl Pts',(16.2103729253055,-18.5139082392468,-12.9886648627694));
#54544=CARTESIAN_POINT('Ctrl Pts',(16.2260880567288,-18.4313924548469,-12.9928435408533));
#54545=CARTESIAN_POINT('Ctrl Pts',(16.2458470513543,-18.3497584337278,-12.9970222189372));
#54546=CARTESIAN_POINT('Ctrl Pts',(16.2659602117581,-18.2666611814494,-13.0012757968227));
#54547=CARTESIAN_POINT('Ctrl Pts',(16.2902636140324,-18.1844780963255,-13.0055293747081));
#54548=CARTESIAN_POINT('Ctrl Pts',(16.3186494198465,-18.1036595170853,-13.0097829525935));
#54549=CARTESIAN_POINT('Ctrl Pts',(16.3464849114244,-18.0244077637083,-13.0139540665715));
#54550=CARTESIAN_POINT('Ctrl Pts',(16.3782457689155,-17.9464685351598,-13.0181251805494));
#54551=CARTESIAN_POINT('Ctrl Pts',(16.4137796304914,-17.8702526002262,-13.0222962945274));
#54552=CARTESIAN_POINT('Ctrl Pts',(16.4493015683369,-17.7940622402856,-13.0264660088478));
#54553=CARTESIAN_POINT('Ctrl Pts',(16.4885938016076,-17.7195944421082,-13.0306357231681));
#54554=CARTESIAN_POINT('Ctrl Pts',(16.5314561548595,-17.6472392517271,-13.0348054374885));
#54555=CARTESIAN_POINT('Ctrl Pts',(16.5743169828848,-17.5748866360543,-13.0389750034325));
#54556=CARTESIAN_POINT('Ctrl Pts',(16.6207474431035,-17.5046468740728,-13.0431445693766));
#54557=CARTESIAN_POINT('Ctrl Pts',(16.6705024900493,-17.4368834941077,-13.0473141353206));
#54558=CARTESIAN_POINT('Ctrl Pts',(16.7220068630664,-17.366737637298,-13.0516302980595));
#54559=CARTESIAN_POINT('Ctrl Pts',(16.7770736453878,-17.2992459668448,-13.0559464607985));
#54560=CARTESIAN_POINT('Ctrl Pts',(16.8353848266788,-17.234775371818,-13.0602626235374));
#54561=CARTESIAN_POINT('Ctrl Pts',(16.8917965273724,-17.1724048996433,-13.0644381877291));
#54562=CARTESIAN_POINT('Ctrl Pts',(16.9512441342268,-17.1128620023875,-13.0686137519207));
#54563=CARTESIAN_POINT('Ctrl Pts',(17.0134027193002,-17.0564407163983,-13.0727893161124));
#54564=CARTESIAN_POINT('Ctrl Pts',(17.078700786738,-16.9971697253824,-13.077175778125));
#54565=CARTESIAN_POINT('Ctrl Pts',(17.146990440611,-16.9413443477726,-13.0815622401375));
#54566=CARTESIAN_POINT('Ctrl Pts',(17.2178583236867,-16.889255610274,-13.0859487021501));
#54567=CARTESIAN_POINT('Ctrl Pts',(17.2887262067624,-16.8371668727754,-13.0903351641627));
#54568=CARTESIAN_POINT('Ctrl Pts',(17.3621717925896,-16.7888150309009,-13.0947216261752));
#54569=CARTESIAN_POINT('Ctrl Pts',(17.4377516489583,-16.7444356832877,-13.0991080881878));
#54570=CARTESIAN_POINT('Ctrl Pts',(17.5098539640989,-16.7020982952443,-13.1032927225808));
#54571=CARTESIAN_POINT('Ctrl Pts',(17.5841668423745,-16.6632182861073,-13.1074773569739));
#54572=CARTESIAN_POINT('Ctrl Pts',(17.6603248069611,-16.6280332231607,-13.1116619913669));
#54573=CARTESIAN_POINT('Ctrl Pts',(17.7363743701116,-16.5928982417961,-13.1158406694509));
#54574=CARTESIAN_POINT('Ctrl Pts',(17.8142633889644,-16.5614479512896,-13.1200193475348));
#54575=CARTESIAN_POINT('Ctrl Pts',(17.8935998508937,-16.5338751915209,-13.1241980256187));
#54576=CARTESIAN_POINT('Ctrl Pts',(17.9743583618848,-16.5058082098496,-13.1284516035042));
#54577=CARTESIAN_POINT('Ctrl Pts',(18.0566163014193,-16.4817593798135,-13.1327051813896));
#54578=CARTESIAN_POINT('Ctrl Pts',(18.1399366350505,-16.461881786255,-13.136958759275));
#54579=CARTESIAN_POINT('Ctrl Pts',(18.221641641428,-16.4423895586354,-13.141129873253));
#54580=CARTESIAN_POINT('Ctrl Pts',(18.3043677482547,-16.4269083873418,-13.145300987231));
#54581=CARTESIAN_POINT('Ctrl Pts',(18.3876870934188,-16.4155325015417,-13.1494721012089));
#54582=CARTESIAN_POINT('Ctrl Pts',(18.470978479972,-16.4041604330299,-13.1536418155293));
#54583=CARTESIAN_POINT('Ctrl Pts',(18.5548622540878,-16.39689097632,-13.1578115298496));
#54584=CARTESIAN_POINT('Ctrl Pts',(18.6389020976076,-16.3937669400618,-13.16198124417));
#54585=CARTESIAN_POINT('Ctrl Pts',(18.7229389506291,-16.3906430149703,-13.1661508101141));
#54586=CARTESIAN_POINT('Ctrl Pts',(18.8071314022655,-16.3916642332765,-13.1703203760581));
#54587=CARTESIAN_POINT('Ctrl Pts',(18.8910411442615,-16.3968213215102,-13.1744899420021));
#54588=CARTESIAN_POINT('Ctrl Pts',(18.9779010492721,-16.4021597266042,-13.1788061047411));
#54589=CARTESIAN_POINT('Ctrl Pts',(19.0644574681809,-16.4119302148937,-13.18312226748));
#54590=CARTESIAN_POINT('Ctrl Pts',(19.1502297723791,-16.4260639801085,-13.1874384302189));
#54591=CARTESIAN_POINT('Ctrl Pts',(19.2332080527898,-16.4397373394081,-13.1916139944106));
#54592=CARTESIAN_POINT('Ctrl Pts',(19.3154520685914,-16.4574939280207,-13.1957895586023));
#54593=CARTESIAN_POINT('Ctrl Pts',(19.3965387044157,-16.4792196892665,-13.1999651227939));
#54594=CARTESIAN_POINT('Ctrl Pts',(19.4817208334502,-16.5020427670648,-13.2043515848065));
#54595=CARTESIAN_POINT('Ctrl Pts',(19.5656250358877,-16.5292463408117,-13.208738046819));
#54596=CARTESIAN_POINT('Ctrl Pts',(19.6477828618953,-16.5606403697255,-13.2131245088315));
#54597=CARTESIAN_POINT('Ctrl Pts',(19.7299406879029,-16.5920343986394,-13.2175109708441));
#54598=CARTESIAN_POINT('Ctrl Pts',(19.8103516376767,-16.6276185783624,-13.2218974328566));
#54599=CARTESIAN_POINT('Ctrl Pts',(19.888577588602,-16.6671475776545,-13.2262838948691));
#54600=CARTESIAN_POINT('Ctrl Pts',(19.9631842212831,-16.704847669447,-13.2304674063032));
#54601=CARTESIAN_POINT('Ctrl Pts',(20.0360812001481,-16.7462759047423,-13.2346509177373));
#54602=CARTESIAN_POINT('Ctrl Pts',(20.1068712604678,-16.7912537163791,-13.2388344291714));
#54603=CARTESIAN_POINT('Ctrl Pts',(20.170910038113,-16.8319419721225,-13.242618957074));
#54604=CARTESIAN_POINT('Ctrl Pts',(20.2332245718103,-16.875534330629,-13.2464034849766));
#54605=CARTESIAN_POINT('Ctrl Pts',(20.293535888361,-16.9218650751948,-13.2501880128791));
#54606=CARTESIAN_POINT('Ctrl Pts',(20.2954167197789,-16.919379410122,-12.4500366865268));
#54607=CARTESIAN_POINT('Ctrl Pts',(20.3656979408681,-16.9725279852605,-12.4544341426114));
#54608=CARTESIAN_POINT('Ctrl Pts',(21.0821531496881,-17.5778644531088,-12.5012235342565));
#54609=CARTESIAN_POINT('Ctrl Pts',(21.7088251808773,-19.5120955140474,-12.590404861462));
#54610=CARTESIAN_POINT('Ctrl Pts',(19.8732647581097,-21.7565262795287,-12.7175806681434));
#54611=CARTESIAN_POINT('Ctrl Pts',(17.0319370527368,-21.4324760457865,-12.8430154491732));
#54612=CARTESIAN_POINT('Ctrl Pts',(16.1727139550341,-19.7651271422422,-12.9260582946424));
#54613=CARTESIAN_POINT('Ctrl Pts',(16.1699654914217,-18.9513691601896,-12.9667092045512));
#54614=CARTESIAN_POINT('Origin',(18.734,-18.952,1.76670989022851));
#54615=CARTESIAN_POINT('',(20.293535888361,-16.9218650751948,-11.6500725313516));
#54616=CARTESIAN_POINT('',(20.293535888361,-16.9218650751948,-11.7167617890113));
#54617=CARTESIAN_POINT('',(20.293535888361,-16.9218650751948,1.76670989022851));
#54618=CARTESIAN_POINT('',(16.1740010233873,-18.9542890482673,-12.2332901098107));
#54619=CARTESIAN_POINT('Ctrl Pts',(20.293535888361,-16.9218650751948,-11.7167617890113));
#54620=CARTESIAN_POINT('Ctrl Pts',(20.360016796482,-16.9729352581854,-11.7209383138016));
#54621=CARTESIAN_POINT('Ctrl Pts',(20.4240745379401,-17.0273421081747,-11.725114838592));
#54622=CARTESIAN_POINT('Ctrl Pts',(20.485358352181,-17.0848246139568,-11.7292913633823));
#54623=CARTESIAN_POINT('Ctrl Pts',(20.5465832917244,-17.1422518969172,-11.7334638758305));
#54624=CARTESIAN_POINT('Ctrl Pts',(20.6050392660196,-17.202748650016,-11.7376363882786));
#54625=CARTESIAN_POINT('Ctrl Pts',(20.6604085786251,-17.2660136453103,-11.7418089007268));
#54626=CARTESIAN_POINT('Ctrl Pts',(20.7157496012222,-17.3292463164316,-11.7459792813007));
#54627=CARTESIAN_POINT('Ctrl Pts',(20.7680067910422,-17.3952440759125,-11.7501496618745));
#54628=CARTESIAN_POINT('Ctrl Pts',(20.816900154276,-17.463669745212,-11.7543200424484));
#54629=CARTESIAN_POINT('Ctrl Pts',(20.8657832032303,-17.5320809798025,-11.7584895432614));
#54630=CARTESIAN_POINT('Ctrl Pts',(20.9113035680159,-17.6029187325087,-11.7626590440744));
#54631=CARTESIAN_POINT('Ctrl Pts',(20.9532231573676,-17.6758148340451,-11.7668285448873));
#54632=CARTESIAN_POINT('Ctrl Pts',(20.9951464783424,-17.7487174246902,-11.7709984168634));
#54633=CARTESIAN_POINT('Ctrl Pts',(21.0334681592267,-17.8236783285432,-11.7751682888395));
#54634=CARTESIAN_POINT('Ctrl Pts',(21.0679955424597,-17.9003038424628,-11.7793381608156));
#54635=CARTESIAN_POINT('Ctrl Pts',(21.102559332555,-17.977010152964,-11.7835124296483));
#54636=CARTESIAN_POINT('Ctrl Pts',(21.1333206472027,-18.0553841579024,-11.7876866984811));
#54637=CARTESIAN_POINT('Ctrl Pts',(21.160134794313,-18.1350116525776,-11.7918609673138));
#54638=CARTESIAN_POINT('Ctrl Pts',(21.1869637585583,-18.2146831483293,-11.796037542791));
#54639=CARTESIAN_POINT('Ctrl Pts',(21.2098410870979,-18.2956090701708,-11.8002141182683));
#54640=CARTESIAN_POINT('Ctrl Pts',(21.2286725247027,-18.3773618577806,-11.8043906937455));
#54641=CARTESIAN_POINT('Ctrl Pts',(21.2475364626071,-18.4592557387125,-11.8085744773795));
#54642=CARTESIAN_POINT('Ctrl Pts',(21.2623404828511,-18.5419788823773,-11.8127582610135));
#54643=CARTESIAN_POINT('Ctrl Pts',(21.2730418541168,-18.6250956362436,-11.8169420446475));
#54644=CARTESIAN_POINT('Ctrl Pts',(21.280709708843,-18.6846512930032,-11.8199398515935));
#54645=CARTESIAN_POINT('Ctrl Pts',(21.2862722940103,-18.7444088953349,-11.8229376585394));
#54646=CARTESIAN_POINT('Ctrl Pts',(21.2897303495758,-18.8042083214207,-11.8259354654853));
#54647=CARTESIAN_POINT('Ctrl Pts',(21.2945574443532,-18.8876822540643,-11.8301200998784));
#54648=CARTESIAN_POINT('Ctrl Pts',(21.295299648515,-18.9715482669722,-11.8343047342714));
#54649=CARTESIAN_POINT('Ctrl Pts',(21.2919120526423,-19.0553727766261,-11.8384893686645));
#54650=CARTESIAN_POINT('Ctrl Pts',(21.288529278593,-19.1390779724659,-11.8426680467484));
#54651=CARTESIAN_POINT('Ctrl Pts',(21.281028398999,-19.2227413266667,-11.8468467248323));
#54652=CARTESIAN_POINT('Ctrl Pts',(21.2694164102339,-19.3059260187056,-11.8510254029163));
#54653=CARTESIAN_POINT('Ctrl Pts',(21.2575962849155,-19.3906017365655,-11.8552789808017));
#54654=CARTESIAN_POINT('Ctrl Pts',(21.2415161896729,-19.4747809821048,-11.8595325586872));
#54655=CARTESIAN_POINT('Ctrl Pts',(21.2212390250856,-19.5580049769524,-11.8637861365726));
#54656=CARTESIAN_POINT('Ctrl Pts',(21.2013549729015,-19.6396155122616,-11.8679572505505));
#54657=CARTESIAN_POINT('Ctrl Pts',(21.1774352498111,-19.7203070376072,-11.8721283645285));
#54658=CARTESIAN_POINT('Ctrl Pts',(21.1495909652079,-19.7996557607932,-11.8762994785064));
#54659=CARTESIAN_POINT('Ctrl Pts',(21.1217560240233,-19.8789778577488,-11.8804691928268));
#54660=CARTESIAN_POINT('Ctrl Pts',(21.0899992889562,-19.9569576137028,-11.8846389071472));
#54661=CARTESIAN_POINT('Ctrl Pts',(21.0544814935982,-20.0331871428518,-11.8888086214675));
#54662=CARTESIAN_POINT('Ctrl Pts',(21.0189649621159,-20.109413959427,-11.8929781874116));
#54663=CARTESIAN_POINT('Ctrl Pts',(20.9796878315025,-20.1838902563956,-11.8971477533556));
#54664=CARTESIAN_POINT('Ctrl Pts',(20.936858101798,-20.2562301113465,-11.9013173192997));
#54665=CARTESIAN_POINT('Ctrl Pts',(20.8925225316333,-20.3311133463566,-11.9056334820386));
#54666=CARTESIAN_POINT('Ctrl Pts',(20.8443801641983,-20.4037066556453,-11.9099496447775));
#54667=CARTESIAN_POINT('Ctrl Pts',(20.7927112772807,-20.4736135766998,-11.9142658075164));
#54668=CARTESIAN_POINT('Ctrl Pts',(20.7427254989198,-20.5412432871539,-11.9184413717081));
#54669=CARTESIAN_POINT('Ctrl Pts',(20.689439760407,-20.6063586052094,-11.9226169358998));
#54670=CARTESIAN_POINT('Ctrl Pts',(20.6331484080957,-20.6686348837268,-11.9267925000914));
#54671=CARTESIAN_POINT('Ctrl Pts',(20.5740139133991,-20.7340565890242,-11.931178962104));
#54672=CARTESIAN_POINT('Ctrl Pts',(20.5115626117393,-20.796344505447,-11.9355654241165));
#54673=CARTESIAN_POINT('Ctrl Pts',(20.4461771444977,-20.8551682599969,-11.9399518861291));
#54674=CARTESIAN_POINT('Ctrl Pts',(20.3807916772561,-20.9139920145469,-11.9443383481416));
#54675=CARTESIAN_POINT('Ctrl Pts',(20.3124725431191,-20.9693513010386,-11.9487248101541));
#54676=CARTESIAN_POINT('Ctrl Pts',(20.2416377781119,-21.0209679383717,-11.9531112721667));
#54677=CARTESIAN_POINT('Ctrl Pts',(20.1740622256448,-21.0702096177069,-11.9572959065597));
#54678=CARTESIAN_POINT('Ctrl Pts',(20.1039459219093,-21.1162287760929,-11.9614805409528));
#54679=CARTESIAN_POINT('Ctrl Pts',(20.0316291334116,-21.1587529612808,-11.9656651753458));
#54680=CARTESIAN_POINT('Ctrl Pts',(19.9594152789112,-21.2012166185545,-11.9698438534297));
#54681=CARTESIAN_POINT('Ctrl Pts',(19.8850075541825,-21.2401949526838,-11.9740225315137));
#54682=CARTESIAN_POINT('Ctrl Pts',(19.8087770431608,-21.2754574038476,-11.9782012095976));
#54683=CARTESIAN_POINT('Ctrl Pts',(19.731180155015,-21.311351909106,-11.9824547874831));
#54684=CARTESIAN_POINT('Ctrl Pts',(19.6516948805992,-21.343395722762,-11.9867083653685));
#54685=CARTESIAN_POINT('Ctrl Pts',(19.5707410268107,-21.3713934062181,-11.9909619432539));
#54686=CARTESIAN_POINT('Ctrl Pts',(19.4913566214465,-21.3988482999475,-11.9951330572319));
#54687=CARTESIAN_POINT('Ctrl Pts',(19.4105605259062,-21.4224123904405,-11.9993041712098));
#54688=CARTESIAN_POINT('Ctrl Pts',(19.3287692237674,-21.4419497124358,-12.0034752851878));
#54689=CARTESIAN_POINT('Ctrl Pts',(19.24700536749,-21.461480478494,-12.0076449995082));
#54690=CARTESIAN_POINT('Ctrl Pts',(19.1642474149188,-21.4769870528098,-12.0118147138285));
#54691=CARTESIAN_POINT('Ctrl Pts',(19.0809253355101,-21.4883838060477,-12.0159844281489));
#54692=CARTESIAN_POINT('Ctrl Pts',(18.9976062210585,-21.4997801537403,-12.0201539940929));
#54693=CARTESIAN_POINT('Ctrl Pts',(18.9137234755862,-21.5070669096296,-12.024323560037));
#54694=CARTESIAN_POINT('Ctrl Pts',(18.8297141852437,-21.5102100763509,-12.028493125981));
#54695=CARTESIAN_POINT('Ctrl Pts',(18.7427512318894,-21.5134637529366,-12.0328092887199));
#54696=CARTESIAN_POINT('Ctrl Pts',(18.6556531965172,-21.5122770220956,-12.0371254514589));
#54697=CARTESIAN_POINT('Ctrl Pts',(18.5689051504098,-21.5066709554537,-12.0414416141978));
#54698=CARTESIAN_POINT('Ctrl Pts',(18.4849829127802,-21.501247505843,-12.0456171783895));
#54699=CARTESIAN_POINT('Ctrl Pts',(18.4013886754049,-21.4916883190585,-12.0497927425811));
#54700=CARTESIAN_POINT('Ctrl Pts',(18.3185547392503,-21.4780651684627,-12.0539683067728));
#54701=CARTESIAN_POINT('Ctrl Pts',(18.2315370578994,-21.4637539449163,-12.0583547687854));
#54702=CARTESIAN_POINT('Ctrl Pts',(18.1453590723583,-21.444957551129,-12.0627412307979));
#54703=CARTESIAN_POINT('Ctrl Pts',(18.0605056905581,-21.4218189033104,-12.0671276928105));
#54704=CARTESIAN_POINT('Ctrl Pts',(17.9756523087579,-21.3986802554919,-12.071514154823));
#54705=CARTESIAN_POINT('Ctrl Pts',(17.8921240580818,-21.371199607226,-12.0759006168356));
#54706=CARTESIAN_POINT('Ctrl Pts',(17.8103811197836,-21.3395778865008,-12.0802870788481));
#54707=CARTESIAN_POINT('Ctrl Pts',(17.7323992952486,-21.3094111280208,-12.0844717132412));
#54708=CARTESIAN_POINT('Ctrl Pts',(17.6557518403844,-21.2753637103368,-12.0886563476342));
#54709=CARTESIAN_POINT('Ctrl Pts',(17.5808520242221,-21.2375742704973,-12.0928409820273));
#54710=CARTESIAN_POINT('Ctrl Pts',(17.5060588186775,-21.1998386192481,-12.0970196601112));
#54711=CARTESIAN_POINT('Ctrl Pts',(17.4330087179883,-21.1583717310105,-12.1011983381951));
#54712=CARTESIAN_POINT('Ctrl Pts',(17.3620964471735,-21.113360830991,-12.1053770162791));
#54713=CARTESIAN_POINT('Ctrl Pts',(17.289913124868,-21.0675431429373,-12.1096305941645));
#54714=CARTESIAN_POINT('Ctrl Pts',(17.2199454771429,-21.018053314544,-12.11388417205));
#54715=CARTESIAN_POINT('Ctrl Pts',(17.1525850704414,-20.9651385497698,-12.1181377499354));
#54716=CARTESIAN_POINT('Ctrl Pts',(17.0865305766668,-20.9132496409654,-12.1223088639133));
#54717=CARTESIAN_POINT('Ctrl Pts',(17.0229835115634,-20.8580677061308,-12.1264799778913));
#54718=CARTESIAN_POINT('Ctrl Pts',(16.9622836350606,-20.7998693466276,-12.1306510918693));
#54719=CARTESIAN_POINT('Ctrl Pts',(16.9016041269875,-20.741690516146,-12.1348208061896));
#54720=CARTESIAN_POINT('Ctrl Pts',(16.8437702418585,-20.6804975893352,-12.13899052051));
#54721=CARTESIAN_POINT('Ctrl Pts',(16.7890867147049,-20.6166057529284,-12.1431602348304));
#54722=CARTESIAN_POINT('Ctrl Pts',(16.7344051334259,-20.5527161900675,-12.1473298007744));
#54723=CARTESIAN_POINT('Ctrl Pts',(16.682873985715,-20.4861282586161,-12.1514993667185));
#54724=CARTESIAN_POINT('Ctrl Pts',(16.6347584444192,-20.4171910767278,-12.1556689326625));
#54725=CARTESIAN_POINT('Ctrl Pts',(16.5849512200484,-20.3458301485675,-12.1599850954014));
#54726=CARTESIAN_POINT('Ctrl Pts',(16.5388045582795,-20.2719521294865,-12.1643012581404));
#54727=CARTESIAN_POINT('Ctrl Pts',(16.496563301095,-20.1959762933404,-12.1686174208793));
#54728=CARTESIAN_POINT('Ctrl Pts',(16.4556980484202,-20.1224753620654,-12.172792985071));
#54729=CARTESIAN_POINT('Ctrl Pts',(16.4184878365308,-20.0470116310055,-12.1769685492626));
#54730=CARTESIAN_POINT('Ctrl Pts',(16.3851063117009,-19.9699874464201,-12.1811441134543));
#54731=CARTESIAN_POINT('Ctrl Pts',(16.350038765409,-19.8890729533789,-12.1855305754669));
#54732=CARTESIAN_POINT('Ctrl Pts',(16.3191970489118,-19.8064367740456,-12.1899170374794));
#54733=CARTESIAN_POINT('Ctrl Pts',(16.2927234637601,-19.7225639970856,-12.1943034994919));
#54734=CARTESIAN_POINT('Ctrl Pts',(16.2662498786084,-19.6386912201256,-12.1986899615045));
#54735=CARTESIAN_POINT('Ctrl Pts',(16.2441444970407,-19.5535824262448,-12.203076423517));
#54736=CARTESIAN_POINT('Ctrl Pts',(16.2264874578015,-19.4677333135615,-12.2074628855296));
#54737=CARTESIAN_POINT('Ctrl Pts',(16.2025156137684,-19.3511814097151,-12.2134181072288));
#54738=CARTESIAN_POINT('Ctrl Pts',(16.1866633864905,-19.2329068373031,-12.219373328928));
#54739=CARTESIAN_POINT('Ctrl Pts',(16.1791211349008,-19.1138455580776,-12.2253285506272));
#54740=CARTESIAN_POINT('Ctrl Pts',(16.1757600463668,-19.060787728371,-12.2279824036753));
#54741=CARTESIAN_POINT('Ctrl Pts',(16.1740486686438,-19.0075739736056,-12.2306362567234));
#54742=CARTESIAN_POINT('Ctrl Pts',(16.174001023388,-18.9542890490546,-12.2332901097715));
#54743=CARTESIAN_POINT('Ctrl Pts',(16.1740010233873,-18.9542890482673,-12.2332901098107));
#54744=CARTESIAN_POINT('Ctrl Pts',(16.1739252094451,-18.869501140071,-12.2375129674107));
#54745=CARTESIAN_POINT('Ctrl Pts',(16.1780663695147,-18.7845778436852,-12.2417358250107));
#54746=CARTESIAN_POINT('Ctrl Pts',(16.1864353355331,-18.6999796032861,-12.2459586826108));
#54747=CARTESIAN_POINT('Ctrl Pts',(16.1945865434513,-18.6175825848873,-12.2500716626647));
#54748=CARTESIAN_POINT('Ctrl Pts',(16.2067481850333,-18.5354944186516,-12.2541846427187));
#54749=CARTESIAN_POINT('Ctrl Pts',(16.2228775801224,-18.4541403888766,-12.2582976227727));
#54750=CARTESIAN_POINT('Ctrl Pts',(16.2389992540557,-18.3728253033474,-12.2624086339395));
#54751=CARTESIAN_POINT('Ctrl Pts',(16.2590848209399,-18.2922441216164,-12.2665196451063));
#54752=CARTESIAN_POINT('Ctrl Pts',(16.2830401055299,-18.2128142346481,-12.2706306562731));
#54753=CARTESIAN_POINT('Ctrl Pts',(16.3069915898917,-18.13339694831,-12.2747410152756));
#54754=CARTESIAN_POINT('Ctrl Pts',(16.3348114354692,-18.0551310480635,-12.2788513742782));
#54755=CARTESIAN_POINT('Ctrl Pts',(16.3663553936721,-17.9784194855451,-12.2829617332808));
#54756=CARTESIAN_POINT('Ctrl Pts',(16.3994039228382,-17.8980489659369,-12.2872681465249));
#54757=CARTESIAN_POINT('Ctrl Pts',(16.4365404963283,-17.8193852938553,-12.2915745597691));
#54758=CARTESIAN_POINT('Ctrl Pts',(16.4775431085385,-17.74286713014,-12.2958809730133));
#54759=CARTESIAN_POINT('Ctrl Pts',(16.5167281737212,-17.6697408322964,-12.2999964933322));
#54760=CARTESIAN_POINT('Ctrl Pts',(16.5594435017452,-17.5985742591835,-12.304112013651));
#54761=CARTESIAN_POINT('Ctrl Pts',(16.6054498638679,-17.5297221375653,-12.3082275339699));
#54762=CARTESIAN_POINT('Ctrl Pts',(16.6514869443888,-17.46082404346,-12.3123458022172));
#54763=CARTESIAN_POINT('Ctrl Pts',(16.7008191449124,-17.394243852655,-12.3164640704645));
#54764=CARTESIAN_POINT('Ctrl Pts',(16.7531665958489,-17.3303036582026,-12.3205823387118));
#54765=CARTESIAN_POINT('Ctrl Pts',(16.8055945346489,-17.2662651512335,-12.3247069390843));
#54766=CARTESIAN_POINT('Ctrl Pts',(16.8610466479906,-17.204875081261,-12.3288315394568));
#54767=CARTESIAN_POINT('Ctrl Pts',(16.9192065009782,-17.1464184992341,-12.3329561398293));
#54768=CARTESIAN_POINT('Ctrl Pts',(16.9271149034353,-17.1384697484517,-12.3335169906232));
#54769=CARTESIAN_POINT('Ctrl Pts',(16.9350733229401,-17.1305751748483,-12.3340778414171));
#54770=CARTESIAN_POINT('Ctrl Pts',(16.9430809195059,-17.122735435449,-12.334638692211));
#54771=CARTESIAN_POINT('Ctrl Pts',(17.0028274053095,-17.0642413698601,-12.338823326604));
#54772=CARTESIAN_POINT('Ctrl Pts',(17.0655538444185,-17.0085686402268,-12.3430079609971));
#54773=CARTESIAN_POINT('Ctrl Pts',(17.1309629349575,-16.9560360303603,-12.3471925953901));
#54774=CARTESIAN_POINT('Ctrl Pts',(17.1962789237522,-16.9035781941616,-12.3513712734741));
#54775=CARTESIAN_POINT('Ctrl Pts',(17.2642696237812,-16.854251885356,-12.355549951558));
#54776=CARTESIAN_POINT('Ctrl Pts',(17.3346011829202,-16.8083388908795,-12.359728629642));
#54777=CARTESIAN_POINT('Ctrl Pts',(17.4061933847103,-16.7616029389742,-12.3639822075274));
#54778=CARTESIAN_POINT('Ctrl Pts',(17.480210846325,-16.7184042096098,-12.3682357854128));
#54779=CARTESIAN_POINT('Ctrl Pts',(17.556266426922,-16.6789967816026,-12.3724893632983));
#54780=CARTESIAN_POINT('Ctrl Pts',(17.630847521679,-16.6403533434846,-12.3766604772762));
#54781=CARTESIAN_POINT('Ctrl Pts',(17.7073879875337,-16.6053557363937,-12.3808315912542));
#54782=CARTESIAN_POINT('Ctrl Pts',(17.7854953736993,-16.5741987101765,-12.3850027052321));
#54783=CARTESIAN_POINT('Ctrl Pts',(17.8635765501771,-16.5430521390004,-12.3891724195525));
#54784=CARTESIAN_POINT('Ctrl Pts',(17.943223175792,-16.5157437595366,-12.3933421338729));
#54785=CARTESIAN_POINT('Ctrl Pts',(18.0240221782539,-16.4924204642605,-12.3975118481933));
#54786=CARTESIAN_POINT('Ctrl Pts',(18.1048183055405,-16.4690979989273,-12.4016814141373));
#54787=CARTESIAN_POINT('Ctrl Pts',(18.186766285919,-16.4497604625988,-12.4058509800813));
#54788=CARTESIAN_POINT('Ctrl Pts',(18.2694385404887,-16.4345046871272,-12.4100205460254));
#54789=CARTESIAN_POINT('Ctrl Pts',(18.3550174495419,-16.41871253741,-12.4143367087643));
#54790=CARTESIAN_POINT('Ctrl Pts',(18.4413719926993,-16.407294614139,-12.4186528715032));
#54791=CARTESIAN_POINT('Ctrl Pts',(18.5280191484753,-16.4003001961819,-12.4229690342421));
#54792=CARTESIAN_POINT('Ctrl Pts',(18.6118437822656,-16.3935336206541,-12.4271445984338));
#54793=CARTESIAN_POINT('Ctrl Pts',(18.6959417854338,-16.3909067522804,-12.4313201626255));
#54794=CARTESIAN_POINT('Ctrl Pts',(18.7798750222018,-16.3924110716097,-12.4354957268172));
#54795=CARTESIAN_POINT('Ctrl Pts',(18.8680475272268,-16.3939913705323,-12.4398821888297));
#54796=CARTESIAN_POINT('Ctrl Pts',(18.9560376012528,-16.4001311167978,-12.4442686508423));
#54797=CARTESIAN_POINT('Ctrl Pts',(19.0433447687657,-16.4107590011891,-12.4486551128548));
#54798=CARTESIAN_POINT('Ctrl Pts',(19.1306519362786,-16.4213868855805,-12.4530415748673));
#54799=CARTESIAN_POINT('Ctrl Pts',(19.2172756387744,-16.4365027334242,-12.4574280368799));
#54800=CARTESIAN_POINT('Ctrl Pts',(19.3027314805895,-16.4559742583486,-12.4618144988924));
#54801=CARTESIAN_POINT('Ctrl Pts',(19.3842631981423,-16.4745516526699,-12.4659995349797));
#54802=CARTESIAN_POINT('Ctrl Pts',(19.4650354649563,-16.4971626268787,-12.4701845710669));
#54803=CARTESIAN_POINT('Ctrl Pts',(19.5446191872091,-16.5237297239952,-12.4743696071542));
#54804=CARTESIAN_POINT('Ctrl Pts',(19.6240693838797,-16.5502522468318,-12.4785476215872));
#54805=CARTESIAN_POINT('Ctrl Pts',(19.7023345681444,-16.5807175510206,-12.4827256360202));
#54806=CARTESIAN_POINT('Ctrl Pts',(19.7789972930805,-16.6149975058947,-12.4869036504532));
#54807=CARTESIAN_POINT('Ctrl Pts',(19.8555857432772,-16.6492442486084,-12.4910776170138));
#54808=CARTESIAN_POINT('Ctrl Pts',(19.9305743987682,-16.6872981181988,-12.4952515835743));
#54809=CARTESIAN_POINT('Ctrl Pts',(20.0035631940899,-16.7289819397467,-12.4994255501349));
#54810=CARTESIAN_POINT('Ctrl Pts',(20.0764986900048,-16.7706353220615,-12.5035964686941));
#54811=CARTESIAN_POINT('Ctrl Pts',(20.1474368294329,-16.8159131614313,-12.5077673872534));
#54812=CARTESIAN_POINT('Ctrl Pts',(20.2160009920398,-16.8645917841512,-12.5119383058127));
#54813=CARTESIAN_POINT('Ctrl Pts',(20.2421989296968,-16.8831915814033,-12.5135319877047));
#54814=CARTESIAN_POINT('Ctrl Pts',(20.2680505442949,-16.9022874066306,-12.5151256695967));
#54815=CARTESIAN_POINT('Ctrl Pts',(20.293535888361,-16.9218650751948,-12.5167193514888));
#54816=CARTESIAN_POINT('',(16.1740007840082,-18.949996472737,-12.1667098902285));
#54817=CARTESIAN_POINT('Ctrl Pts',(16.1763510013672,-18.9499800105097,-12.1667107986216));
#54818=CARTESIAN_POINT('Ctrl Pts',(16.1742902547169,-18.6667985525942,-12.1807663462203));
#54819=CARTESIAN_POINT('Ctrl Pts',(16.3483939296849,-17.5319993745477,-12.2372138293795));
#54820=CARTESIAN_POINT('Ctrl Pts',(17.9381456496072,-16.0798453637573,-12.3316557920145));
#54821=CARTESIAN_POINT('Ctrl Pts',(19.6881796352386,-16.4601701745045,-12.4120422070509));
#54822=CARTESIAN_POINT('Ctrl Pts',(20.2954167197789,-16.919379410122,-12.4500366865268));
#54823=CARTESIAN_POINT('Ctrl Pts',(20.293535888361,-16.9218650751948,-11.6500725313516));
#54824=CARTESIAN_POINT('Ctrl Pts',(20.3602862242945,-16.9731422308047,-11.65424767163));
#54825=CARTESIAN_POINT('Ctrl Pts',(20.4244786682837,-17.0276947507719,-11.6584228119083));
#54826=CARTESIAN_POINT('Ctrl Pts',(20.4857877623676,-17.0852274815556,-11.6625979521867));
#54827=CARTESIAN_POINT('Ctrl Pts',(20.5471067980569,-17.1427695415867,-11.6667737694869));
#54828=CARTESIAN_POINT('Ctrl Pts',(20.6055412419491,-17.2032924338565,-11.6709495867872));
#54829=CARTESIAN_POINT('Ctrl Pts',(20.6608038266511,-17.2664653626809,-11.6751254040874));
#54830=CARTESIAN_POINT('Ctrl Pts',(20.716166721374,-17.3297529600073,-11.679308801133));
#54831=CARTESIAN_POINT('Ctrl Pts',(20.7683459651374,-17.3956998448477,-11.6834921981786));
#54832=CARTESIAN_POINT('Ctrl Pts',(20.8170955367815,-17.4639432186099,-11.6876755952242));
#54833=CARTESIAN_POINT('Ctrl Pts',(20.8656447850406,-17.5319061643976,-11.6918418017134));
#54834=CARTESIAN_POINT('Ctrl Pts',(20.9107923290493,-17.6021463354618,-11.6960080082027));
#54835=CARTESIAN_POINT('Ctrl Pts',(20.9523407266399,-17.6742815566288,-11.700174214692));
#54836=CARTESIAN_POINT('Ctrl Pts',(20.9940729004966,-17.7467358452539,-11.704358849085));
#54837=CARTESIAN_POINT('Ctrl Pts',(21.0323293070735,-17.8213716700562,-11.7085434834781));
#54838=CARTESIAN_POINT('Ctrl Pts',(21.0668754476401,-17.8978215778161,-11.7127281178711));
#54839=CARTESIAN_POINT('Ctrl Pts',(21.1013724160515,-17.9741626685949,-11.7169067959551));
#54840=CARTESIAN_POINT('Ctrl Pts',(21.1321694205718,-18.0523122977904,-11.721085474039));
#54841=CARTESIAN_POINT('Ctrl Pts',(21.1590769104972,-18.1318768518244,-11.725264152123));
#54842=CARTESIAN_POINT('Ctrl Pts',(21.1864666978414,-18.2128675433073,-11.7295177300084));
#54843=CARTESIAN_POINT('Ctrl Pts',(21.2098259193362,-18.2953239658209,-11.7337713078938));
#54844=CARTESIAN_POINT('Ctrl Pts',(21.2290051549003,-18.3788078184229,-11.7380248857793));
#54845=CARTESIAN_POINT('Ctrl Pts',(21.2478125635577,-18.4606731736369,-11.7421959997572));
#54846=CARTESIAN_POINT('Ctrl Pts',(21.2626005065823,-18.5435260079664,-11.7463671137352));
#54847=CARTESIAN_POINT('Ctrl Pts',(21.2732783407021,-18.6269376852954,-11.7505382277131));
#54848=CARTESIAN_POINT('Ctrl Pts',(21.2839525917715,-18.7103213730303,-11.7547079420335));
#54849=CARTESIAN_POINT('Ctrl Pts',(21.2905194146576,-18.7942630754073,-11.7588776563539));
#54850=CARTESIAN_POINT('Ctrl Pts',(21.2929396556081,-18.8783261311161,-11.7630473706742));
#54851=CARTESIAN_POINT('Ctrl Pts',(21.295359810436,-18.9623861955009,-11.7672169366183));
#54852=CARTESIAN_POINT('Ctrl Pts',(21.2936336643145,-19.0465671447647,-11.7713865025623));
#54853=CARTESIAN_POINT('Ctrl Pts',(21.2877741604491,-19.1304307636668,-11.7755560685064));
#54854=CARTESIAN_POINT('Ctrl Pts',(21.2817086436562,-19.2172429239524,-11.7798722312453));
#54855=CARTESIAN_POINT('Ctrl Pts',(21.2712137402018,-19.3037144978784,-11.7841883939842));
#54856=CARTESIAN_POINT('Ctrl Pts',(21.2563622783627,-19.3893654498163,-11.7885045567231));
#54857=CARTESIAN_POINT('Ctrl Pts',(21.2419946013309,-19.4722263310037,-11.7926801209148));
#54858=CARTESIAN_POINT('Ctrl Pts',(21.2235499863025,-19.554318783463,-11.7968556851065));
#54859=CARTESIAN_POINT('Ctrl Pts',(21.2011460288053,-19.6352206616827,-11.8010312492982));
#54860=CARTESIAN_POINT('Ctrl Pts',(21.1776105006753,-19.7202087014454,-11.8054177113107));
#54861=CARTESIAN_POINT('Ctrl Pts',(21.1497053305465,-19.8038821804658,-11.8098041733232));
#54862=CARTESIAN_POINT('Ctrl Pts',(21.1176244749812,-19.8857742565903,-11.8141906353358));
#54863=CARTESIAN_POINT('Ctrl Pts',(21.0855436194159,-19.9676663327147,-11.8185770973483));
#54864=CARTESIAN_POINT('Ctrl Pts',(21.0492873869464,-20.0477765087051,-11.8229635593609));
#54865=CARTESIAN_POINT('Ctrl Pts',(21.0091047687183,-20.1256687315232,-11.8273500213734));
#54866=CARTESIAN_POINT('Ctrl Pts',(20.9707710123197,-20.1999770177056,-11.8315346557664));
#54867=CARTESIAN_POINT('Ctrl Pts',(20.9287215623263,-20.2725435578142,-11.8357192901595));
#54868=CARTESIAN_POINT('Ctrl Pts',(20.8831384590297,-20.3429722800686,-11.8399039245525));
#54869=CARTESIAN_POINT('Ctrl Pts',(20.8376202376386,-20.4133007557544,-11.8440826026365));
#54870=CARTESIAN_POINT('Ctrl Pts',(20.7885786013675,-20.481497074883,-11.8482612807204));
#54871=CARTESIAN_POINT('Ctrl Pts',(20.7362419167442,-20.5471887997452,-11.8524399588044));
#54872=CARTESIAN_POINT('Ctrl Pts',(20.6829671346629,-20.6140580015636,-11.8566935366898));
#54873=CARTESIAN_POINT('Ctrl Pts',(20.6262782358932,-20.6783315077606,-11.8609471145753));
#54874=CARTESIAN_POINT('Ctrl Pts',(20.5664628839088,-20.7396464357072,-11.8652006924607));
#54875=CARTESIAN_POINT('Ctrl Pts',(20.5078071692427,-20.7997726541292,-11.8693718064387));
#54876=CARTESIAN_POINT('Ctrl Pts',(20.4461454804006,-20.8570536417645,-11.8735429204166));
#54877=CARTESIAN_POINT('Ctrl Pts',(20.3817891690389,-20.9111811693659,-11.8777140343946));
#54878=CARTESIAN_POINT('Ctrl Pts',(20.317454453059,-20.9652905339527,-11.8818837487149));
#54879=CARTESIAN_POINT('Ctrl Pts',(20.2504272621008,-21.0162482441942,-11.8860534630353));
#54880=CARTESIAN_POINT('Ctrl Pts',(20.1810535660396,-21.0637850214954,-11.8902231773557));
#54881=CARTESIAN_POINT('Ctrl Pts',(20.1116823385923,-21.1113201072339,-11.8943927432997));
#54882=CARTESIAN_POINT('Ctrl Pts',(20.0399651520291,-21.1554342427326,-11.8985623092438));
#54883=CARTESIAN_POINT('Ctrl Pts',(19.9662774819301,-21.1959011135806,-11.9027318751878));
#54884=CARTESIAN_POINT('Ctrl Pts',(19.8899990442537,-21.2377907496864,-11.9070480379267));
#54885=CARTESIAN_POINT('Ctrl Pts',(19.811609442817,-21.2757716196387,-11.9113642006656));
#54886=CARTESIAN_POINT('Ctrl Pts',(19.7315517321809,-21.309645126312,-11.9156803634045));
#54887=CARTESIAN_POINT('Ctrl Pts',(19.6541018930483,-21.3424152070683,-11.9198559275962));
#54888=CARTESIAN_POINT('Ctrl Pts',(19.5750914116572,-21.3713412922627,-11.9240314917879));
#54889=CARTESIAN_POINT('Ctrl Pts',(19.4949388978056,-21.3962937617656,-11.9282070559796));
#54890=CARTESIAN_POINT('Ctrl Pts',(19.4107380710239,-21.4225065211842,-11.9325935179921));
#54891=CARTESIAN_POINT('Ctrl Pts',(19.3252773774555,-21.4443335563955,-11.9369799800047));
#54892=CARTESIAN_POINT('Ctrl Pts',(19.239054342481,-21.4616852613707,-11.9413664420172));
#54893=CARTESIAN_POINT('Ctrl Pts',(19.1528313075064,-21.4790369663458,-11.9457529040297));
#54894=CARTESIAN_POINT('Ctrl Pts',(19.0658465162267,-21.4919133313661,-11.9501393660423));
#54895=CARTESIAN_POINT('Ctrl Pts',(18.9786013944249,-21.5002876913421,-11.9545258280548));
#54896=CARTESIAN_POINT('Ctrl Pts',(18.8953705500055,-21.5082767346017,-11.9587104624479));
#54897=CARTESIAN_POINT('Ctrl Pts',(18.8115930039276,-21.5121986934545,-11.9628950968409));
#54898=CARTESIAN_POINT('Ctrl Pts',(18.7277003248363,-21.5119922488345,-11.967079731234));
#54899=CARTESIAN_POINT('Ctrl Pts',(18.6439270565898,-21.5117860980629,-11.9712584093179));
#54900=CARTESIAN_POINT('Ctrl Pts',(18.560039436939,-21.507463217065,-11.9754370874018));
#54901=CARTESIAN_POINT('Ctrl Pts',(18.4764742375282,-21.4990140324826,-11.9796157654858));
#54902=CARTESIAN_POINT('Ctrl Pts',(18.391411191975,-21.4904134023389,-11.9838693433712));
#54903=CARTESIAN_POINT('Ctrl Pts',(18.3066827190521,-21.4775370395473,-11.9881229212567));
#54904=CARTESIAN_POINT('Ctrl Pts',(18.2227496524054,-21.460430402081,-11.9923764991421));
#54905=CARTESIAN_POINT('Ctrl Pts',(18.1404437920376,-21.4436554101629,-11.99654761312));
#54906=CARTESIAN_POINT('Ctrl Pts',(18.0589032436853,-21.4228128002076,-12.000718727098));
#54907=CARTESIAN_POINT('Ctrl Pts',(17.9785557081133,-21.3979975310404,-12.004889841076));
#54908=CARTESIAN_POINT('Ctrl Pts',(17.898235133933,-21.3731905888765,-12.0090595553963));
#54909=CARTESIAN_POINT('Ctrl Pts',(17.819107216658,-21.3444137706279,-12.0132292697167));
#54910=CARTESIAN_POINT('Ctrl Pts',(17.7415856439041,-21.3118122268127,-12.0173989840371));
#54911=CARTESIAN_POINT('Ctrl Pts',(17.6640668297004,-21.2792118431003,-12.0215685499811));
#54912=CARTESIAN_POINT('Ctrl Pts',(17.5881546700965,-21.2427871835461,-12.0257381159252));
#54913=CARTESIAN_POINT('Ctrl Pts',(17.5142426975068,-21.2027314639944,-12.0299076818692));
#54914=CARTESIAN_POINT('Ctrl Pts',(17.4377320711412,-21.1612674347574,-12.0342238446081));
#54915=CARTESIAN_POINT('Ctrl Pts',(17.3633653656329,-21.1159125099135,-12.0385400073471));
#54916=CARTESIAN_POINT('Ctrl Pts',(17.2915493867665,-21.0669317313763,-12.042856170086));
#54917=CARTESIAN_POINT('Ctrl Pts',(17.222072805858,-21.0195464965481,-12.0470317342777));
#54918=CARTESIAN_POINT('Ctrl Pts',(17.1549836708369,-20.968768326667,-12.0512072984694));
#54919=CARTESIAN_POINT('Ctrl Pts',(17.0906175572636,-20.914879045409,-12.055382862661));
#54920=CARTESIAN_POINT('Ctrl Pts',(17.0230004643097,-20.8582679446643,-12.0597693246736));
#54921=CARTESIAN_POINT('Ctrl Pts',(16.9583891293619,-20.7982235859986,-12.0641557866861));
#54922=CARTESIAN_POINT('Ctrl Pts',(16.8971281979621,-20.735115807478,-12.0685422486987));
#54923=CARTESIAN_POINT('Ctrl Pts',(16.8358672665623,-20.6720080289574,-12.0729287107112));
#54924=CARTESIAN_POINT('Ctrl Pts',(16.7779570635865,-20.6058373172987,-12.0773151727238));
#54925=CARTESIAN_POINT('Ctrl Pts',(16.7236914224212,-20.5370108589259,-12.0817016347363));
#54926=CARTESIAN_POINT('Ctrl Pts',(16.6719732357611,-20.4714154002739,-12.0858821780095));
#54927=CARTESIAN_POINT('Ctrl Pts',(16.62336875941,-20.403158891998,-12.0900627212828));
#54928=CARTESIAN_POINT('Ctrl Pts',(16.5781640651477,-20.3325692383938,-12.094243264556));
#54929=CARTESIAN_POINT('Ctrl Pts',(16.5330221281564,-20.2620775837719,-12.0984180040186));
#54930=CARTESIAN_POINT('Ctrl Pts',(16.4912708487477,-20.1892595981085,-12.1025927434812));
#54931=CARTESIAN_POINT('Ctrl Pts',(16.4531558825332,-20.1144758542942,-12.1067674829437));
#54932=CARTESIAN_POINT('Ctrl Pts',(16.4150823671081,-20.0397734392997,-12.1109376822935));
#54933=CARTESIAN_POINT('Ctrl Pts',(16.380637519025,-19.9631099194743,-12.1151078816432));
#54934=CARTESIAN_POINT('Ctrl Pts',(16.3500227648594,-19.8848732723855,-12.119278080993));
#54935=CARTESIAN_POINT('Ctrl Pts',(16.319430601241,-19.8066943559144,-12.1234452031635));
#54936=CARTESIAN_POINT('Ctrl Pts',(16.2926630858425,-19.7269450449961,-12.1276123253341));
#54937=CARTESIAN_POINT('Ctrl Pts',(16.2698743296479,-19.6460350716728,-12.1317794475046));
#54938=CARTESIAN_POINT('Ctrl Pts',(16.2470959536797,-19.5651619526576,-12.1359446715605));
#54939=CARTESIAN_POINT('Ctrl Pts',(16.2282928589745,-19.4831296648129,-12.1401098956164));
#54940=CARTESIAN_POINT('Ctrl Pts',(16.2135694674,-19.4003636139762,-12.1442751196724));
#54941=CARTESIAN_POINT('Ctrl Pts',(16.1988435352848,-19.3175832817472,-12.1484410624432));
#54942=CARTESIAN_POINT('Ctrl Pts',(16.1881988016354,-19.2340693856754,-12.1526070052141));
#54943=CARTESIAN_POINT('Ctrl Pts',(16.1816884763611,-19.1502571216887,-12.156772947985));
#54944=CARTESIAN_POINT('Ctrl Pts',(16.1765121589547,-19.0836185341113,-12.1600852620661));
#54945=CARTESIAN_POINT('Ctrl Pts',(16.1739485082683,-19.0167915973248,-12.1633975761473));
#54946=CARTESIAN_POINT('Ctrl Pts',(16.1740007840082,-18.949996472737,-12.1667098902285));
#54947=CARTESIAN_POINT('Origin',(18.734,-18.952,1.76670989022851));
#54948=CARTESIAN_POINT('',(20.2922820154253,-16.9234654489967,-10.8502164909775));
#54949=CARTESIAN_POINT('',(20.2948050591539,-16.920183071726,-10.9165936719733));
#54950=CARTESIAN_POINT('',(20.293535888361,-16.9218650751948,1.76670989022851));
#54951=CARTESIAN_POINT('',(16.1739804747524,-18.9506989546656,-11.4332901033215));
#54952=CARTESIAN_POINT('Ctrl Pts',(20.2948050591539,-16.920183071726,-10.9165936719733));
#54953=CARTESIAN_POINT('Ctrl Pts',(20.3968578832778,-16.9970801053588,-10.9229640542206));
#54954=CARTESIAN_POINT('Ctrl Pts',(21.1313725981362,-17.6446400837689,-10.9717263720284));
#54955=CARTESIAN_POINT('Ctrl Pts',(21.6797113984698,-19.6491907408466,-11.0628806253967));
#54956=CARTESIAN_POINT('Ctrl Pts',(19.742230629931,-21.8062532419297,-11.1900564320781));
#54957=CARTESIAN_POINT('Ctrl Pts',(16.9631832264668,-21.35816637253,-11.3135258905595));
#54958=CARTESIAN_POINT('Ctrl Pts',(16.1754043811927,-19.7256331452917,-11.3946034134805));
#54959=CARTESIAN_POINT('Ctrl Pts',(16.1705865782758,-18.9507193134542,-11.433289000841));
#54960=CARTESIAN_POINT('Ctrl Pts',(16.1740003306697,-18.950698835557,-11.4332901097715));
#54961=CARTESIAN_POINT('Ctrl Pts',(16.174038011382,-18.8765632322752,-11.436996088328));
#54962=CARTESIAN_POINT('Ctrl Pts',(16.1772957565522,-18.8025118189363,-11.4407020668845));
#54963=CARTESIAN_POINT('Ctrl Pts',(16.1837535357011,-18.7287446051466,-11.444408045441));
#54964=CARTESIAN_POINT('Ctrl Pts',(16.1910453870482,-18.6454497843057,-11.448592679834));
#54965=CARTESIAN_POINT('Ctrl Pts',(16.2024358975503,-18.5623575749321,-11.4527773142271));
#54966=CARTESIAN_POINT('Ctrl Pts',(16.217906819526,-18.4799034980302,-11.4569619486201));
#54967=CARTESIAN_POINT('Ctrl Pts',(16.2333557205591,-18.3975667843009,-11.4611406267041));
#54968=CARTESIAN_POINT('Ctrl Pts',(16.2528734125179,-18.3158668471442,-11.465319304788));
#54969=CARTESIAN_POINT('Ctrl Pts',(16.2763898192684,-18.2352349062878,-11.469497982872));
#54970=CARTESIAN_POINT('Ctrl Pts',(16.3003277407088,-18.1531576958409,-11.4737515607574));
#54971=CARTESIAN_POINT('Ctrl Pts',(16.3284090988417,-18.0721876262597,-11.4780051386428));
#54972=CARTESIAN_POINT('Ctrl Pts',(16.3605053261112,-17.9927695620856,-11.4822587165282));
#54973=CARTESIAN_POINT('Ctrl Pts',(16.3919793053844,-17.9148911720571,-11.4864298305062));
#54974=CARTESIAN_POINT('Ctrl Pts',(16.4273136905277,-17.8385055933013,-11.4906009444841));
#54975=CARTESIAN_POINT('Ctrl Pts',(16.4663372697809,-17.7640161019714,-11.4947720584621));
#54976=CARTESIAN_POINT('Ctrl Pts',(16.5053477542952,-17.6895516063097,-11.4989417727825));
#54977=CARTESIAN_POINT('Ctrl Pts',(16.5480447610381,-17.6169823416312,-11.5031114871028));
#54978=CARTESIAN_POINT('Ctrl Pts',(16.5942102750742,-17.5466886704001,-11.5072812014232));
#54979=CARTESIAN_POINT('Ctrl Pts',(16.6403741463431,-17.4763975005194,-11.5114507673673));
#54980=CARTESIAN_POINT('Ctrl Pts',(16.6900060262586,-17.4083821471394,-11.5156203333113));
#54981=CARTESIAN_POINT('Ctrl Pts',(16.7428443053793,-17.3429944065419,-11.5197898992553));
#54982=CARTESIAN_POINT('Ctrl Pts',(16.7975403132107,-17.2753077136495,-11.5241060619943));
#54983=CARTESIAN_POINT('Ctrl Pts',(16.8556720579014,-17.2104372553887,-11.5284222247332));
#54984=CARTESIAN_POINT('Ctrl Pts',(16.9169048877879,-17.1487348078625,-11.5327383874721));
#54985=CARTESIAN_POINT('Ctrl Pts',(16.9761430646814,-17.0890423110745,-11.5369139516638));
#54986=CARTESIAN_POINT('Ctrl Pts',(17.0382830139764,-17.0323148814136,-11.5410895158555));
#54987=CARTESIAN_POINT('Ctrl Pts',(17.1029865459476,-16.9788312001503,-11.5452650800471));
#54988=CARTESIAN_POINT('Ctrl Pts',(17.1709580995006,-16.9226461852919,-11.5496515420597));
#54989=CARTESIAN_POINT('Ctrl Pts',(17.2417585461137,-16.8700415621994,-11.5540380040722));
#54990=CARTESIAN_POINT('Ctrl Pts',(17.3149615008575,-16.8212889126042,-11.5584244660848));
#54991=CARTESIAN_POINT('Ctrl Pts',(17.3881644556012,-16.772536263009,-11.5628109280973));
#54992=CARTESIAN_POINT('Ctrl Pts',(17.4637693807619,-16.7276358177823,-11.5671973901098));
#54993=CARTESIAN_POINT('Ctrl Pts',(17.5413224142637,-16.6868023979171,-11.5715838521224));
#54994=CARTESIAN_POINT('Ctrl Pts',(17.615307117733,-16.6478477842295,-11.5757684865154));
#54995=CARTESIAN_POINT('Ctrl Pts',(17.6913399834857,-16.6124491640088,-11.5799531209085));
#54996=CARTESIAN_POINT('Ctrl Pts',(17.7690449301558,-16.5808269331021,-11.5841377553015));
#54997=CARTESIAN_POINT('Ctrl Pts',(17.8466392734524,-16.549249712527,-11.5883164333855));
#54998=CARTESIAN_POINT('Ctrl Pts',(17.9259005477808,-16.5214383763015,-11.5924951114694));
#54999=CARTESIAN_POINT('Ctrl Pts',(18.0064282347098,-16.4975674125468,-11.5966737895534));
#55000=CARTESIAN_POINT('Ctrl Pts',(18.0883993225526,-16.4732685789225,-11.6009273674388));
#55001=CARTESIAN_POINT('Ctrl Pts',(18.1716822438314,-16.4530529941954,-11.6051809453242));
#55002=CARTESIAN_POINT('Ctrl Pts',(18.2558333466885,-16.4370533501362,-11.6094345232097));
#55003=CARTESIAN_POINT('Ctrl Pts',(18.3383530162095,-16.4213638903979,-11.6136056371876));
#55004=CARTESIAN_POINT('Ctrl Pts',(18.4217070321717,-16.4097284515022,-11.6177767511656));
#55005=CARTESIAN_POINT('Ctrl Pts',(18.5054636294716,-16.4022213571869,-11.6219478651435));
#55006=CARTESIAN_POINT('Ctrl Pts',(18.5891921214364,-16.3947167819496,-11.6261175794639));
#55007=CARTESIAN_POINT('Ctrl Pts',(18.6733224686331,-16.3913378410871,-11.6302872937843));
#55008=CARTESIAN_POINT('Ctrl Pts',(18.7574168390734,-16.3921071015279,-11.6344570081047));
#55009=CARTESIAN_POINT('Ctrl Pts',(18.8415082170751,-16.3928763345952,-11.6386265740487));
#55010=CARTESIAN_POINT('Ctrl Pts',(18.9255631608599,-16.3977934704174,-11.6427961399927));
#55011=CARTESIAN_POINT('Ctrl Pts',(19.009144261199,-16.4068289575101,-11.6469657059368));
#55012=CARTESIAN_POINT('Ctrl Pts',(19.0956639699175,-16.4161821211824,-11.6512818686757));
#55013=CARTESIAN_POINT('Ctrl Pts',(19.1816753701876,-16.4299485702282,-11.6555980314146));
#55014=CARTESIAN_POINT('Ctrl Pts',(19.2667015333782,-16.4480373252909,-11.6599141941535));
#55015=CARTESIAN_POINT('Ctrl Pts',(19.348957978246,-16.46553684106,-11.6640897583452));
#55016=CARTESIAN_POINT('Ctrl Pts',(19.4302919452566,-16.4870812228023,-11.6682653225369));
#55017=CARTESIAN_POINT('Ctrl Pts',(19.5102860518794,-16.5125369513646,-11.6724408867286));
#55018=CARTESIAN_POINT('Ctrl Pts',(19.5943204706598,-16.5392783882613,-11.6768273487411));
#55019=CARTESIAN_POINT('Ctrl Pts',(19.6768755727334,-16.570336474695,-11.6812138107537));
#55020=CARTESIAN_POINT('Ctrl Pts',(19.7574922067679,-16.605499690457,-11.6856002727662));
#55021=CARTESIAN_POINT('Ctrl Pts',(19.8381088408023,-16.640662906219,-11.6899867347787));
#55022=CARTESIAN_POINT('Ctrl Pts',(19.9167865216171,-16.6799309241433,-11.6943731967913));
#55023=CARTESIAN_POINT('Ctrl Pts',(19.9930989518199,-16.7230383965788,-11.6987596588038));
#55024=CARTESIAN_POINT('Ctrl Pts',(20.0658940459174,-16.7641589912696,-11.7029439432528));
#55025=CARTESIAN_POINT('Ctrl Pts',(20.1368080586058,-16.8089259475303,-11.7071282277017));
#55026=CARTESIAN_POINT('Ctrl Pts',(20.2054522028094,-16.8571423879301,-11.7113125121506));
#55027=CARTESIAN_POINT('Ctrl Pts',(20.2352510809046,-16.8780734643726,-11.7131289377709));
#55028=CARTESIAN_POINT('Ctrl Pts',(20.2646224661193,-16.8996539802127,-11.7149453633911));
#55029=CARTESIAN_POINT('Ctrl Pts',(20.293535888361,-16.9218650751948,-11.7167617890113));
#55030=CARTESIAN_POINT('',(16.1740004874608,-18.9535798097909,-11.3667098902285));
#55031=CARTESIAN_POINT('Ctrl Pts',(16.1740004874608,-18.9535798097909,-11.3667098902285));
#55032=CARTESIAN_POINT('Ctrl Pts',(16.1739481146197,-18.8687123476393,-11.3709134538372));
#55033=CARTESIAN_POINT('Ctrl Pts',(16.1781202862138,-18.7838299700766,-11.3751170174459));
#55034=CARTESIAN_POINT('Ctrl Pts',(16.1864949217896,-18.699377996817,-11.3793205810546));
#55035=CARTESIAN_POINT('Ctrl Pts',(16.1948707822013,-18.6149136719983,-11.3835247594573));
#55036=CARTESIAN_POINT('Ctrl Pts',(16.2074502833288,-18.5308803238368,-11.3877289378599));
#55037=CARTESIAN_POINT('Ctrl Pts',(16.2241595327126,-18.447717510946,-11.3919331162626));
#55038=CARTESIAN_POINT('Ctrl Pts',(16.2408759290274,-18.3645191274036,-11.3961390928892));
#55039=CARTESIAN_POINT('Ctrl Pts',(16.2617254950327,-18.2821924593937,-11.4003450695159));
#55040=CARTESIAN_POINT('Ctrl Pts',(16.2865836343726,-18.2011650425965,-11.4045510461425));
#55041=CARTESIAN_POINT('Ctrl Pts',(16.3114761780105,-18.1200254817903,-11.408762843948));
#55042=CARTESIAN_POINT('Ctrl Pts',(16.3403882340966,-18.0401891906195,-11.4129746417534));
#55043=CARTESIAN_POINT('Ctrl Pts',(16.3731460171586,-17.9620664306621,-11.4171864395589));
#55044=CARTESIAN_POINT('Ctrl Pts',(16.4059305542806,-17.8838798659902,-11.4214016772397));
#55045=CARTESIAN_POINT('Ctrl Pts',(16.4425668768385,-17.8074100228066,-11.4256169149205));
#55046=CARTESIAN_POINT('Ctrl Pts',(16.4828349986458,-17.7330430127859,-11.4298321526013));
#55047=CARTESIAN_POINT('Ctrl Pts',(16.5231739006091,-17.6585452862497,-11.4340547994973));
#55048=CARTESIAN_POINT('Ctrl Pts',(16.5671571084147,-17.5861581518398,-11.4382774463933));
#55049=CARTESIAN_POINT('Ctrl Pts',(16.6145212917447,-17.5162388759782,-11.4425000932893));
#55050=CARTESIAN_POINT('Ctrl Pts',(16.6269438222717,-17.4979006660113,-11.4436075959693));
#55051=CARTESIAN_POINT('Ctrl Pts',(16.6395987151329,-17.4797320374711,-11.4447150986492));
#55052=CARTESIAN_POINT('Ctrl Pts',(16.6524807786036,-17.4617390393098,-11.4458226013291));
#55053=CARTESIAN_POINT('Ctrl Pts',(16.7011549053849,-17.3937535433782,-11.4500072357222));
#55054=CARTESIAN_POINT('Ctrl Pts',(16.7532538754926,-17.3280286903786,-11.4541918701152));
#55055=CARTESIAN_POINT('Ctrl Pts',(16.8085402991528,-17.2649300724589,-11.4583765045082));
#55056=CARTESIAN_POINT('Ctrl Pts',(16.8637480294321,-17.2019212676117,-11.4625551825922));
#55057=CARTESIAN_POINT('Ctrl Pts',(16.9221339008883,-17.141531615807,-11.4667338606761));
#55058=CARTESIAN_POINT('Ctrl Pts',(16.9834181011139,-17.0840966258148,-11.4709125387601));
#55059=CARTESIAN_POINT('Ctrl Pts',(17.0458007765844,-17.0256321549048,-11.4751661166455));
#55060=CARTESIAN_POINT('Ctrl Pts',(17.1111864272471,-16.9702297043272,-11.4794196945309));
#55061=CARTESIAN_POINT('Ctrl Pts',(17.1792379481544,-16.9182067553114,-11.4836732724164));
#55062=CARTESIAN_POINT('Ctrl Pts',(17.2459701575374,-16.8671923726767,-11.4878443863943));
#55063=CARTESIAN_POINT('Ctrl Pts',(17.3152654110889,-16.8194279167438,-11.4920155003723));
#55064=CARTESIAN_POINT('Ctrl Pts',(17.386771066055,-16.7751733648402,-11.4961866143502));
#55065=CARTESIAN_POINT('Ctrl Pts',(17.4582527266079,-16.7309336629788,-11.5003563286706));
#55066=CARTESIAN_POINT('Ctrl Pts',(17.5319429246537,-16.6902017679485,-11.504526042991));
#55067=CARTESIAN_POINT('Ctrl Pts',(17.6074603942082,-16.6531941107213,-11.5086957573114));
#55068=CARTESIAN_POINT('Ctrl Pts',(17.6829751765272,-16.6161877703853,-11.5128653232554));
#55069=CARTESIAN_POINT('Ctrl Pts',(17.7603166876029,-16.5829056060342,-11.5170348891994));
#55070=CARTESIAN_POINT('Ctrl Pts',(17.8390806772783,-16.5535172700602,-11.5212044551435));
#55071=CARTESIAN_POINT('Ctrl Pts',(17.9206139116647,-16.5230956764479,-11.5255206178824));
#55072=CARTESIAN_POINT('Ctrl Pts',(18.0036710203271,-16.4968470041693,-11.5298367806213));
#55073=CARTESIAN_POINT('Ctrl Pts',(18.0877848913437,-16.4749037093112,-11.5341529433602));
#55074=CARTESIAN_POINT('Ctrl Pts',(18.1691587618592,-16.453675214975,-11.5383285075519));
#55075=CARTESIAN_POINT('Ctrl Pts',(18.2515211332007,-16.4364759603011,-11.5425040717436));
#55076=CARTESIAN_POINT('Ctrl Pts',(18.3344390537291,-16.4233736831602,-11.5466796359353));
#55077=CARTESIAN_POINT('Ctrl Pts',(18.4215449613046,-16.4096096411485,-11.5510660979478));
#55078=CARTESIAN_POINT('Ctrl Pts',(18.5092634338795,-16.4003673913994,-11.5554525599604));
#55079=CARTESIAN_POINT('Ctrl Pts',(18.5970892183628,-16.3956636688668,-11.5598390219729));
#55080=CARTESIAN_POINT('Ctrl Pts',(18.6849150028461,-16.3909599463343,-11.5642254839854));
#55081=CARTESIAN_POINT('Ctrl Pts',(18.7728475188787,-16.3907946760441,-11.568611945998));
#55082=CARTESIAN_POINT('Ctrl Pts',(18.8603867536229,-16.3951217493771,-11.5729984080105));
#55083=CARTESIAN_POINT('Ctrl Pts',(18.9438873685615,-16.3992491933197,-11.5771825007379));
#55084=CARTESIAN_POINT('Ctrl Pts',(19.0273409554117,-16.4074789682949,-11.5813665934652));
#55085=CARTESIAN_POINT('Ctrl Pts',(19.1103117838484,-16.4198093592036,-11.5855506861926));
#55086=CARTESIAN_POINT('Ctrl Pts',(19.1931709965617,-16.4321231627704,-11.5897291503087));
#55087=CARTESIAN_POINT('Ctrl Pts',(19.2755482894343,-16.448526562281,-11.5939076144249));
#55088=CARTESIAN_POINT('Ctrl Pts',(19.357010161509,-16.4689659006255,-11.598086078541));
#55089=CARTESIAN_POINT('Ctrl Pts',(19.4414693002971,-16.4901572735956,-11.6024182829419));
#55090=CARTESIAN_POINT('Ctrl Pts',(19.5249438451359,-16.5156873315821,-11.6067504873428));
#55091=CARTESIAN_POINT('Ctrl Pts',(19.6069591096031,-16.5454376399185,-11.6110826917437));
#55092=CARTESIAN_POINT('Ctrl Pts',(19.6859209486914,-16.5740803453337,-11.6152536083288));
#55093=CARTESIAN_POINT('Ctrl Pts',(19.763529765532,-16.6066344601364,-11.6194245249139));
#55094=CARTESIAN_POINT('Ctrl Pts',(19.8393764673876,-16.6429432953377,-11.6235954414991));
#55095=CARTESIAN_POINT('Ctrl Pts',(19.9151926442948,-16.6792375178362,-11.6277646794744));
#55096=CARTESIAN_POINT('Ctrl Pts',(19.9892477021866,-16.719283257044,-11.6319339174498));
#55097=CARTESIAN_POINT('Ctrl Pts',(20.0611538617777,-16.7628762878337,-11.6361031554252));
#55098=CARTESIAN_POINT('Ctrl Pts',(20.1330612502713,-16.8064700636442,-11.6402724646544));
#55099=CARTESIAN_POINT('Ctrl Pts',(20.202819273287,-16.8536110146999,-11.6444417738836));
#55100=CARTESIAN_POINT('Ctrl Pts',(20.2700670848392,-16.9040503153462,-11.6486110831128));
#55101=CARTESIAN_POINT('Ctrl Pts',(20.2779244372492,-16.9099437318209,-11.6490982325257));
#55102=CARTESIAN_POINT('Ctrl Pts',(20.2857475543659,-16.9158821298114,-11.6495853819387));
#55103=CARTESIAN_POINT('Ctrl Pts',(20.293535888361,-16.9218650751948,-11.6500725313516));
#55104=CARTESIAN_POINT('Ctrl Pts',(20.2922820154255,-16.9234654489969,-10.8502164909775));
#55105=CARTESIAN_POINT('Ctrl Pts',(20.7519191282237,-17.2828443540149,-10.8791841188528));
#55106=CARTESIAN_POINT('Ctrl Pts',(21.5989576167214,-18.5500198638012,-10.9505436822886));
#55107=CARTESIAN_POINT('Ctrl Pts',(20.9146849414325,-21.0515011378533,-11.0642951812848));
#55108=CARTESIAN_POINT('Ctrl Pts',(18.1490151951601,-21.9220310806025,-11.1914709879662));
#55109=CARTESIAN_POINT('Ctrl Pts',(16.3822353344203,-20.4522479494082,-11.2922755723059));
#55110=CARTESIAN_POINT('Ctrl Pts',(16.1753927157401,-19.2766421922516,-11.350688221085));
#55111=CARTESIAN_POINT('Ctrl Pts',(16.177204683354,-18.953597107844,-11.3667089343037));
#55112=CARTESIAN_POINT('Origin',(18.734,-18.952,1.76670989022851));
#55113=CARTESIAN_POINT('',(20.293535888361,-16.9218650751948,-10.0501312781553));
#55114=CARTESIAN_POINT('',(20.293535888361,-16.9218650751948,-10.1166694971161));
#55115=CARTESIAN_POINT('',(20.293535888361,-16.9218650751948,1.76670989022851));
#55116=CARTESIAN_POINT('',(16.1740004874608,-18.9504201902088,-10.6332901097715));
#55117=CARTESIAN_POINT('Ctrl Pts',(20.293535888361,-16.9218650751947,-10.1166694971161));
#55118=CARTESIAN_POINT('Ctrl Pts',(20.3602256419765,-16.9730956918787,-10.120839657233));
#55119=CARTESIAN_POINT('Ctrl Pts',(20.4243735084243,-17.0276044555347,-10.1250098173499));
#55120=CARTESIAN_POINT('Ctrl Pts',(20.4856520344282,-17.0851001231229,-10.1291799774668));
#55121=CARTESIAN_POINT('Ctrl Pts',(20.5469978537159,-17.1426589298323,-10.1333547170634));
#55122=CARTESIAN_POINT('Ctrl Pts',(20.6054677076776,-17.2032108717433,-10.1375294566601));
#55123=CARTESIAN_POINT('Ctrl Pts',(20.6607708315928,-17.2664276454204,-10.1417041962567));
#55124=CARTESIAN_POINT('Ctrl Pts',(20.7161082334552,-17.329683602078,-10.1458815234378));
#55125=CARTESIAN_POINT('Ctrl Pts',(20.7682747131804,-17.3956073175892,-10.1500588506188));
#55126=CARTESIAN_POINT('Ctrl Pts',(20.8170211514923,-17.4638390939029,-10.1542361777999));
#55127=CARTESIAN_POINT('Ctrl Pts',(20.8658480308291,-17.5321834658074,-10.1584203983765));
#55128=CARTESIAN_POINT('Ctrl Pts',(20.9112433552803,-17.6028431144115,-10.1626046189532));
#55129=CARTESIAN_POINT('Ctrl Pts',(20.9530027200995,-17.6754315810772,-10.1667888395298));
#55130=CARTESIAN_POINT('Ctrl Pts',(20.9725011699955,-17.7093248786989,-10.1687425525621));
#55131=CARTESIAN_POINT('Ctrl Pts',(20.9912075876463,-17.7436383769395,-10.1706962655943));
#55132=CARTESIAN_POINT('Ctrl Pts',(21.0091047687182,-17.7783312684767,-10.1726499786266));
#55133=CARTESIAN_POINT('Ctrl Pts',(21.0474385251168,-17.8526395546591,-10.1768346130197));
#55134=CARTESIAN_POINT('Ctrl Pts',(21.0821992629535,-17.9289661561369,-10.1810192474127));
#55135=CARTESIAN_POINT('Ctrl Pts',(21.1131697431269,-18.0069331593007,-10.1852038818058));
#55136=CARTESIAN_POINT('Ctrl Pts',(21.1440961406553,-18.0847891860861,-10.1893825598897));
#55137=CARTESIAN_POINT('Ctrl Pts',(21.1712428282378,-18.1642805528131,-10.1935612379737));
#55138=CARTESIAN_POINT('Ctrl Pts',(21.1944386775071,-18.2450052940602,-10.1977399160576));
#55139=CARTESIAN_POINT('Ctrl Pts',(21.2180502957041,-18.327176968278,-10.2019934939431));
#55140=CARTESIAN_POINT('Ctrl Pts',(21.2375678238505,-18.4106262399203,-10.2062470718285));
#55141=CARTESIAN_POINT('Ctrl Pts',(21.252862289631,-18.4949083616223,-10.2105006497139));
#55142=CARTESIAN_POINT('Ctrl Pts',(21.2678602423477,-18.5775565099321,-10.2146717636919));
#55143=CARTESIAN_POINT('Ctrl Pts',(21.2787973301571,-18.6610050301441,-10.2188428776698));
#55144=CARTESIAN_POINT('Ctrl Pts',(21.2856028472,-18.7448215499602,-10.2230139916478));
#55145=CARTESIAN_POINT('Ctrl Pts',(21.2924060805859,-18.8286099443337,-10.2271837059682));
#55146=CARTESIAN_POINT('Ctrl Pts',(21.2950804593957,-18.9127656349242,-10.2313534202885));
#55147=CARTESIAN_POINT('Ctrl Pts',(21.2936070835643,-18.9968506161339,-10.2355231346089));
#55148=CARTESIAN_POINT('Ctrl Pts',(21.2921337601619,-19.0809326052393,-10.239692700553));
#55149=CARTESIAN_POINT('Ctrl Pts',(21.2865129844866,-19.1649434300193,-10.243862266497));
#55150=CARTESIAN_POINT('Ctrl Pts',(21.2767779695195,-19.2484459440205,-10.2480318324411));
#55151=CARTESIAN_POINT('Ctrl Pts',(21.2667006834357,-19.3348843034021,-10.25234799518));
#55152=CARTESIAN_POINT('Ctrl Pts',(21.2522145228801,-19.4207774186565,-10.2566641579189));
#55153=CARTESIAN_POINT('Ctrl Pts',(21.2334144574579,-19.5056491396638,-10.2609803206578));
#55154=CARTESIAN_POINT('Ctrl Pts',(21.2152268021893,-19.5877561732863,-10.2651558848495));
#55155=CARTESIAN_POINT('Ctrl Pts',(21.1930021468738,-19.668906892756,-10.2693314490412));
#55156=CARTESIAN_POINT('Ctrl Pts',(21.166877500828,-19.7486850481621,-10.2735070132329));
#55157=CARTESIAN_POINT('Ctrl Pts',(21.1394333610159,-19.8324926085431,-10.2778934752454));
#55158=CARTESIAN_POINT('Ctrl Pts',(21.1076851096662,-19.9147847597334,-10.2822799372579));
#55159=CARTESIAN_POINT('Ctrl Pts',(21.0718481041567,-19.9951041376061,-10.2866663992705));
#55160=CARTESIAN_POINT('Ctrl Pts',(21.0360110986472,-20.0754235154788,-10.291052861283));
#55161=CARTESIAN_POINT('Ctrl Pts',(20.9960856701951,-20.15376963761,-10.2954393232956));
#55162=CARTESIAN_POINT('Ctrl Pts',(20.9523407266399,-20.2297184433712,-10.2998257853081));
#55163=CARTESIAN_POINT('Ctrl Pts',(20.9106085527831,-20.3021727319963,-10.3040104197011));
#55164=CARTESIAN_POINT('Ctrl Pts',(20.8652452879882,-20.3727151532424,-10.3081950540942));
#55165=CARTESIAN_POINT('Ctrl Pts',(20.8164511103895,-20.440958485935,-10.3123796884872));
#55166=CARTESIAN_POINT('Ctrl Pts',(20.7677263852629,-20.5091046826904,-10.3165583665712));
#55167=CARTESIAN_POINT('Ctrl Pts',(20.7155807127377,-20.5749579200271,-10.3207370446551));
#55168=CARTESIAN_POINT('Ctrl Pts',(20.6602594535816,-20.6381567298112,-10.3249157227391));
#55169=CARTESIAN_POINT('Ctrl Pts',(20.603946600614,-20.7024883328402,-10.3291693006245));
#55170=CARTESIAN_POINT('Ctrl Pts',(20.5443434371028,-20.7640689932949,-10.33342287851));
#55171=CARTESIAN_POINT('Ctrl Pts',(20.4817541149309,-20.8225495325551,-10.3376764563954));
#55172=CARTESIAN_POINT('Ctrl Pts',(20.4203782089023,-20.8798963124463,-10.3418475703733));
#55173=CARTESIAN_POINT('Ctrl Pts',(20.3561312476116,-20.9342617737267,-10.3460186843513));
#55174=CARTESIAN_POINT('Ctrl Pts',(20.2893385159965,-20.9853524290338,-10.3501897983292));
#55175=CARTESIAN_POINT('Ctrl Pts',(20.2225681973275,-21.0364259403781,-10.3543595126496));
#55176=CARTESIAN_POINT('Ctrl Pts',(20.1532541699938,-21.0842265489053,-10.35852922697));
#55177=CARTESIAN_POINT('Ctrl Pts',(20.0817544971403,-21.1285012785289,-10.3626989412904));
#55178=CARTESIAN_POINT('Ctrl Pts',(20.0102573685523,-21.1727744326675,-10.3668685072344));
#55179=CARTESIAN_POINT('Ctrl Pts',(19.9365751406472,-21.2135217158936,-10.3710380731785));
#55180=CARTESIAN_POINT('Ctrl Pts',(19.8610933619694,-21.2505344359841,-10.3752076391225));
#55181=CARTESIAN_POINT('Ctrl Pts',(19.78295773707,-21.2888484776529,-10.3795238018614));
#55182=CARTESIAN_POINT('Ctrl Pts',(19.7028941360643,-21.3231602233057,-10.3838399646003));
#55183=CARTESIAN_POINT('Ctrl Pts',(19.6213543310965,-21.3532917963222,-10.3881561273392));
#55184=CARTESIAN_POINT('Ctrl Pts',(19.5424706766991,-21.382441836517,-10.3923316915309));
#55185=CARTESIAN_POINT('Ctrl Pts',(19.4622059796066,-21.4076797638284,-10.3965072557226));
#55186=CARTESIAN_POINT('Ctrl Pts',(19.3809844006654,-21.4288954732277,-10.4006828199143));
#55187=CARTESIAN_POINT('Ctrl Pts',(19.2956605128578,-21.4511827376731,-10.4050692819268));
#55188=CARTESIAN_POINT('Ctrl Pts',(19.2092811104196,-21.469030663203,-10.4094557439394));
#55189=CARTESIAN_POINT('Ctrl Pts',(19.122347333066,-21.4823727687636,-10.4138422059519));
#55190=CARTESIAN_POINT('Ctrl Pts',(19.0354135557123,-21.4957148743243,-10.4182286679644));
#55191=CARTESIAN_POINT('Ctrl Pts',(18.947925988367,-21.50455117729,-10.422615129977));
#55192=CARTESIAN_POINT('Ctrl Pts',(18.8603867536229,-21.5088782506229,-10.4270015919895));
#55193=CARTESIAN_POINT('Ctrl Pts',(18.7768753288337,-21.5130062288976,-10.4311862263825));
#55194=CARTESIAN_POINT('Ctrl Pts',(18.693006041295,-21.5130461767751,-10.4353708607756));
#55195=CARTESIAN_POINT('Ctrl Pts',(18.6092128353628,-21.5089568169099,-10.4395554951686));
#55196=CARTESIAN_POINT('Ctrl Pts',(18.5255388986877,-21.5048732777423,-10.4437341732526));
#55197=CARTESIAN_POINT('Ctrl Pts',(18.4419412840716,-21.4966721277451,-10.4479128513365));
#55198=CARTESIAN_POINT('Ctrl Pts',(18.3588567381415,-21.4843640206499,-10.4520915294204));
#55199=CARTESIAN_POINT('Ctrl Pts',(18.2742829614372,-21.4718352995807,-10.4563451073059));
#55200=CARTESIAN_POINT('Ctrl Pts',(18.1902413094004,-21.4550509150074,-10.4605986851913));
#55201=CARTESIAN_POINT('Ctrl Pts',(18.1071900176372,-21.4340776067662,-10.4648522630767));
#55202=CARTESIAN_POINT('Ctrl Pts',(18.0257488372261,-21.4135109070313,-10.4690233770547));
#55203=CARTESIAN_POINT('Ctrl Pts',(17.9452604262034,-21.3889163729565,-10.4731944910326));
#55204=CARTESIAN_POINT('Ctrl Pts',(17.8661476315627,-21.360408658554,-10.4773656050106));
#55205=CARTESIAN_POINT('Ctrl Pts',(17.7870613839843,-21.3319105101903,-10.481535319331));
#55206=CARTESIAN_POINT('Ctrl Pts',(17.7093502684721,-21.2995019451709,-10.4857050336513));
#55207=CARTESIAN_POINT('Ctrl Pts',(17.6334208106696,-21.2633471067784,-10.4898747479717));
#55208=CARTESIAN_POINT('Ctrl Pts',(17.5574940547628,-21.2271935549301,-10.4940443139158));
#55209=CARTESIAN_POINT('Ctrl Pts',(17.4833492454958,-21.1872941933041,-10.4982138798598));
#55210=CARTESIAN_POINT('Ctrl Pts',(17.4113705501161,-21.1438602460695,-10.5023834458039));
#55211=CARTESIAN_POINT('Ctrl Pts',(17.3368611726025,-21.0988992148319,-10.5066996085428));
#55212=CARTESIAN_POINT('Ctrl Pts',(17.2646735157618,-21.0501506938737,-10.5110157712817));
#55213=CARTESIAN_POINT('Ctrl Pts',(17.1952016813753,-20.9978982708331,-10.5153319340206));
#55214=CARTESIAN_POINT('Ctrl Pts',(17.1279928846869,-20.947347964977,-10.5195074982123));
#55215=CARTESIAN_POINT('Ctrl Pts',(17.0633260236107,-20.8935188682644,-10.523683062404));
#55216=CARTESIAN_POINT('Ctrl Pts',(17.0015232692729,-20.8367080350784,-10.5278586265957));
#55217=CARTESIAN_POINT('Ctrl Pts',(16.9365990047356,-20.7770278217632,-10.5322450886082));
#55218=CARTESIAN_POINT('Ctrl Pts',(16.8748361916356,-20.7140571577261,-10.5366315506207));
#55219=CARTESIAN_POINT('Ctrl Pts',(16.816561987441,-20.6481814372271,-10.5410180126333));
#55220=CARTESIAN_POINT('Ctrl Pts',(16.7582877832464,-20.5823057167281,-10.5454044746458));
#55221=CARTESIAN_POINT('Ctrl Pts',(16.7035024899564,-20.513525441,-10.5497909366584));
#55222=CARTESIAN_POINT('Ctrl Pts',(16.6524807786035,-20.4422609606901,-10.5541773986709));
#55223=CARTESIAN_POINT('Ctrl Pts',(16.6033728384837,-20.3736695367859,-10.5583993290636));
#55224=CARTESIAN_POINT('Ctrl Pts',(16.55756917535,-20.302523084569,-10.5626212594563));
#55225=CARTESIAN_POINT('Ctrl Pts',(16.5153433201942,-20.2291697370175,-10.5668431898491));
#55226=CARTESIAN_POINT('Ctrl Pts',(16.4731798646836,-20.1559247880487,-10.5710588812454));
#55227=CARTESIAN_POINT('Ctrl Pts',(16.4345839361667,-20.0804798079436,-10.5752745726417));
#55228=CARTESIAN_POINT('Ctrl Pts',(16.3997870211452,-20.0032134746785,-10.579490264038));
#55229=CARTESIAN_POINT('Ctrl Pts',(16.3650317212897,-19.9260395476307,-10.583700913703));
#55230=CARTESIAN_POINT('Ctrl Pts',(16.3340665899187,-19.8470490030815,-10.587911563368));
#55231=CARTESIAN_POINT('Ctrl Pts',(16.3070776023617,-19.7666457364042,-10.5921222130329));
#55232=CARTESIAN_POINT('Ctrl Pts',(16.2801155537111,-19.686322723796,-10.5963286598616));
#55233=CARTESIAN_POINT('Ctrl Pts',(16.2571218975387,-19.6045902181233,-10.6005351066902));
#55234=CARTESIAN_POINT('Ctrl Pts',(16.2382342921444,-19.5218715043693,-10.6047415535189));
#55235=CARTESIAN_POINT('Ctrl Pts',(16.2193575415102,-19.439200329293,-10.6089455828907));
#55236=CARTESIAN_POINT('Ctrl Pts',(16.2045822501753,-19.3555445100533,-10.6131496122625));
#55237=CARTESIAN_POINT('Ctrl Pts',(16.1939957867901,-19.271340878805,-10.6173536416343));
#55238=CARTESIAN_POINT('Ctrl Pts',(16.1834116610727,-19.1871558411241,-10.6215567426862));
#55239=CARTESIAN_POINT('Ctrl Pts',(16.1770145819502,-19.1024236771961,-10.6257598437382));
#55240=CARTESIAN_POINT('Ctrl Pts',(16.1748403468597,-19.0175886403178,-10.6299629447901));
#55241=CARTESIAN_POINT('Ctrl Pts',(16.1742666403856,-18.9952035679304,-10.6310719997839));
#55242=CARTESIAN_POINT('Ctrl Pts',(16.1739866695752,-18.9728113543428,-10.6321810547777));
#55243=CARTESIAN_POINT('Ctrl Pts',(16.1740004874608,-18.9504201902088,-10.6332901097715));
#55244=CARTESIAN_POINT('Ctrl Pts',(16.1772048604514,-18.9504028912009,-10.6332910657491));
#55245=CARTESIAN_POINT('Ctrl Pts',(16.1753928930938,-18.6273578295265,-10.6493117789502));
#55246=CARTESIAN_POINT('Ctrl Pts',(16.3822354976306,-17.4517521542537,-10.7077244277117));
#55247=CARTESIAN_POINT('Ctrl Pts',(18.037362949687,-16.0748525964386,-10.8021586297865));
#55248=CARTESIAN_POINT('Ctrl Pts',(19.7177437303012,-16.4853660561861,-10.8805721186601));
#55249=CARTESIAN_POINT('Ctrl Pts',(20.2948050591539,-16.920183071726,-10.9165936719733));
#55250=CARTESIAN_POINT('',(16.1739802850659,-18.9533010441961,-10.5667098967402));
#55251=CARTESIAN_POINT('Ctrl Pts',(16.1705864007212,-18.9532806854788,-10.5667109992167));
#55252=CARTESIAN_POINT('Ctrl Pts',(16.1754042043383,-18.178366800346,-10.6053965865579));
#55253=CARTESIAN_POINT('Ctrl Pts',(16.9631831042392,-16.5458334607307,-10.6864741094597));
#55254=CARTESIAN_POINT('Ctrl Pts',(19.090228029654,-16.2028738910185,-10.7809759400466));
#55255=CARTESIAN_POINT('Ctrl Pts',(20.0792749286077,-16.7569204692939,-10.8367921832923));
#55256=CARTESIAN_POINT('Ctrl Pts',(20.2922820154255,-16.9234654489969,-10.8502164909775));
#55257=CARTESIAN_POINT('Ctrl Pts',(20.293535888361,-16.9218650751948,-10.0501312781553));
#55258=CARTESIAN_POINT('Ctrl Pts',(20.3598785012909,-16.972829020757,-10.0543142412582));
#55259=CARTESIAN_POINT('Ctrl Pts',(20.4238373170522,-17.0271382723338,-10.0584972043611));
#55260=CARTESIAN_POINT('Ctrl Pts',(20.4850560926825,-17.0845411489729,-10.0626801674639));
#55261=CARTESIAN_POINT('Ctrl Pts',(20.5461929679461,-17.1418672302726,-10.0668575344697));
#55262=CARTESIAN_POINT('Ctrl Pts',(20.6045967518193,-17.2022784029154,-10.0710349014755));
#55263=CARTESIAN_POINT('Ctrl Pts',(20.6599429831436,-17.2654818039286,-10.0752122684813));
#55264=CARTESIAN_POINT('Ctrl Pts',(20.7152315991736,-17.3286194103528,-10.079385286858));
#55265=CARTESIAN_POINT('Ctrl Pts',(20.7674686870318,-17.3945431235226,-10.0835583052348));
#55266=CARTESIAN_POINT('Ctrl Pts',(20.8163664800914,-17.4629231575933,-10.0877313236115));
#55267=CARTESIAN_POINT('Ctrl Pts',(20.8652367031686,-17.5312646370337,-10.0919019891204));
#55268=CARTESIAN_POINT('Ctrl Pts',(20.9107711025747,-17.6020593143187,-10.0960726546294));
#55269=CARTESIAN_POINT('Ctrl Pts',(20.9527228017081,-17.674945134624,-10.1002433201383));
#55270=CARTESIAN_POINT('Ctrl Pts',(20.9946634319104,-17.7478117240485,-10.1044128852196));
#55271=CARTESIAN_POINT('Ctrl Pts',(21.0330230101449,-17.8227679620443,-10.1085824503009));
#55272=CARTESIAN_POINT('Ctrl Pts',(21.0675992713509,-17.8994248526825,-10.1127520153822));
#55273=CARTESIAN_POINT('Ctrl Pts',(21.1021767816142,-17.9760845125284,-10.1169217310878));
#55274=CARTESIAN_POINT('Ctrl Pts',(21.1329705155016,-18.0544445271115,-10.1210914467934));
#55275=CARTESIAN_POINT('Ctrl Pts',(21.1598258291851,-18.1340947203628,-10.125261162499));
#55276=CARTESIAN_POINT('Ctrl Pts',(21.1867086002934,-18.2138263496091,-10.1294351414077));
#55277=CARTESIAN_POINT('Ctrl Pts',(21.2096447612378,-18.2948503552936,-10.1336091203163));
#55278=CARTESIAN_POINT('Ctrl Pts',(21.2285293388216,-18.3767405995915,-10.137783099225));
#55279=CARTESIAN_POINT('Ctrl Pts',(21.2474234560288,-18.4586722110889,-10.1419591866365));
#55280=CARTESIAN_POINT('Ctrl Pts',(21.2622618321363,-18.5414704795095,-10.1461352740481));
#55281=CARTESIAN_POINT('Ctrl Pts',(21.2729909705675,-18.6247006700641,-10.1503113614597));
#55282=CARTESIAN_POINT('Ctrl Pts',(21.283739223649,-18.7080791405565,-10.1544948888396));
#55283=CARTESIAN_POINT('Ctrl Pts',(21.2903635759395,-18.7918906111061,-10.1586784162195));
#55284=CARTESIAN_POINT('Ctrl Pts',(21.2928626078116,-18.8756969571784,-10.1628619435994));
#55285=CARTESIAN_POINT('Ctrl Pts',(21.2950932319719,-18.9505021096975,-10.1665961405712));
#55286=CARTESIAN_POINT('Ctrl Pts',(21.294037851978,-19.0253029473734,-10.170330337543));
#55287=CARTESIAN_POINT('Ctrl Pts',(21.2897303495757,-19.0997916785801,-10.1740645345148));
#55288=CARTESIAN_POINT('Ctrl Pts',(21.2849032547983,-19.1832656112237,-10.1782491689078));
#55289=CARTESIAN_POINT('Ctrl Pts',(21.2759733033623,-19.2666581465938,-10.1824338033009));
#55290=CARTESIAN_POINT('Ctrl Pts',(21.262945864237,-19.3495334146438,-10.1866184376939));
#55291=CARTESIAN_POINT('Ctrl Pts',(21.2499369680589,-19.4322907200076,-10.1907971157779));
#55292=CARTESIAN_POINT('Ctrl Pts',(21.232842239734,-19.514531769942,-10.1949757938618));
#55293=CARTESIAN_POINT('Ctrl Pts',(21.2117189811603,-19.595823462137,-10.1991544719458));
#55294=CARTESIAN_POINT('Ctrl Pts',(21.1902171033577,-19.6785722494913,-10.2034080498312));
#55295=CARTESIAN_POINT('Ctrl Pts',(21.1645408797954,-19.7603368285348,-10.2076616277166));
#55296=CARTESIAN_POINT('Ctrl Pts',(21.1348056750072,-19.840668729535,-10.2119152056021));
#55297=CARTESIAN_POINT('Ctrl Pts',(21.1056469451873,-19.9194432398795,-10.21608631958));
#55298=CARTESIAN_POINT('Ctrl Pts',(21.0725853792787,-19.9968396756824,-10.220257433558));
#55299=CARTESIAN_POINT('Ctrl Pts',(21.0357801964354,-20.0724498771912,-10.2244285475359));
#55300=CARTESIAN_POINT('Ctrl Pts',(20.9989873639267,-20.1480347069666,-10.2285982618563));
#55301=CARTESIAN_POINT('Ctrl Pts',(20.9584536105076,-20.2218340795557,-10.2327679761767));
#55302=CARTESIAN_POINT('Ctrl Pts',(20.9143856152224,-20.2934613557353,-10.236937690497));
#55303=CARTESIAN_POINT('Ctrl Pts',(20.8703191880656,-20.3650860831091,-10.2411072564411));
#55304=CARTESIAN_POINT('Ctrl Pts',(20.8227190108796,-20.4345384763813,-10.2452768223851));
#55305=CARTESIAN_POINT('Ctrl Pts',(20.7718361823766,-20.5014591617067,-10.2494463883292));
#55306=CARTESIAN_POINT('Ctrl Pts',(20.7191643763941,-20.5707326957726,-10.2537625510681));
#55307=CARTESIAN_POINT('Ctrl Pts',(20.662975107358,-20.6372927599322,-10.258078713807));
#55308=CARTESIAN_POINT('Ctrl Pts',(20.6035924848957,-20.7007778419289,-10.2623948765459));
#55309=CARTESIAN_POINT('Ctrl Pts',(20.5461442451141,-20.7621949040571,-10.2665704407376));
#55310=CARTESIAN_POINT('Ctrl Pts',(20.4857078751412,-20.8207339487951,-10.2707460049293));
#55311=CARTESIAN_POINT('Ctrl Pts',(20.4226131812577,-20.8761064222342,-10.274921569121));
#55312=CARTESIAN_POINT('Ctrl Pts',(20.3563317243795,-20.9342756276711,-10.2793080311335));
#55313=CARTESIAN_POINT('Ctrl Pts',(20.2871168004274,-20.9889496060668,-10.283694493146));
#55314=CARTESIAN_POINT('Ctrl Pts',(20.2153865821741,-21.0398442935608,-10.2880809551586));
#55315=CARTESIAN_POINT('Ctrl Pts',(20.1436563639209,-21.0907389810548,-10.2924674171711));
#55316=CARTESIAN_POINT('Ctrl Pts',(20.0694113820225,-21.1378541309858,-10.2968538791837));
#55317=CARTESIAN_POINT('Ctrl Pts',(19.9930989518198,-21.1809616034213,-10.3012403411962));
#55318=CARTESIAN_POINT('Ctrl Pts',(19.9202977696528,-21.2220856371494,-10.3054249755892));
#55319=CARTESIAN_POINT('Ctrl Pts',(19.845344231219,-21.2597157589185,-10.3096096099823));
#55320=CARTESIAN_POINT('Ctrl Pts',(19.7686077403709,-21.2936205549928,-10.3137942443753));
#55321=CARTESIAN_POINT('Ctrl Pts',(19.6919804744194,-21.3274770917864,-10.3179729224593));
#55322=CARTESIAN_POINT('Ctrl Pts',(19.6135757141378,-21.3576186510692,-10.3221516005432));
#55323=CARTESIAN_POINT('Ctrl Pts',(19.5337886464593,-21.3838589846031,-10.3263302786272));
#55324=CARTESIAN_POINT('Ctrl Pts',(19.4525714529346,-21.4105696572571,-10.3305838565126));
#55325=CARTESIAN_POINT('Ctrl Pts',(19.369922328658,-21.43323763244,-10.334837434398));
#55326=CARTESIAN_POINT('Ctrl Pts',(19.2862808103367,-21.4517171653077,-10.3390910122835));
#55327=CARTESIAN_POINT('Ctrl Pts',(19.2042608460611,-21.4698384363709,-10.3432621262614));
#55328=CARTESIAN_POINT('Ctrl Pts',(19.1212870932382,-21.4839321143086,-10.3474332402394));
#55329=CARTESIAN_POINT('Ctrl Pts',(19.0377889319356,-21.4939111480997,-10.3516043542173));
#55330=CARTESIAN_POINT('Ctrl Pts',(18.9543187892475,-21.5038868333295,-10.3557740685377));
#55331=CARTESIAN_POINT('Ctrl Pts',(18.8703250439617,-21.5097505619763,-10.3599437828581));
#55332=CARTESIAN_POINT('Ctrl Pts',(18.7862446699246,-21.5114668379302,-10.3641134971784));
#55333=CARTESIAN_POINT('Ctrl Pts',(18.702167287828,-21.5131830528116,-10.3682830631225));
#55334=CARTESIAN_POINT('Ctrl Pts',(18.6180037430636,-21.510752099899,-10.3724526290665));
#55335=CARTESIAN_POINT('Ctrl Pts',(18.5341921271335,-21.5041905912256,-10.3766221950106));
#55336=CARTESIAN_POINT('Ctrl Pts',(18.44743379818,-21.4973983880018,-10.3809383577495));
#55337=CARTESIAN_POINT('Ctrl Pts',(18.3610531319648,-21.4861798052051,-10.3852545204884));
#55338=CARTESIAN_POINT('Ctrl Pts',(18.2755295374792,-21.4706116880131,-10.3895706832273));
#55339=CARTESIAN_POINT('Ctrl Pts',(18.1927918650886,-21.4555507006011,-10.393746247419));
#55340=CARTESIAN_POINT('Ctrl Pts',(18.1108567316687,-21.4364193523527,-10.3979218116107));
#55341=CARTESIAN_POINT('Ctrl Pts',(18.0301452832767,-21.413338769399,-10.4020973758024));
#55342=CARTESIAN_POINT('Ctrl Pts',(17.9453572914997,-21.3890924410691,-10.4064838378149));
#55343=CARTESIAN_POINT('Ctrl Pts',(17.8619204024431,-21.3604876310562,-10.4108702998275));
#55344=CARTESIAN_POINT('Ctrl Pts',(17.7802998178502,-21.3277221981047,-10.41525676184));
#55345=CARTESIAN_POINT('Ctrl Pts',(17.6986792332574,-21.2949567651532,-10.4196432238525));
#55346=CARTESIAN_POINT('Ctrl Pts',(17.6188754477654,-21.258031021948,-10.4240296858651));
#55347=CARTESIAN_POINT('Ctrl Pts',(17.5413224142635,-21.2171976020828,-10.4284161478776));
#55348=CARTESIAN_POINT('Ctrl Pts',(17.4673377107943,-21.1782429883953,-10.4326007822707));
#55349=CARTESIAN_POINT('Ctrl Pts',(17.3951258047344,-21.135587395429,-10.4367854166637));
#55350=CARTESIAN_POINT('Ctrl Pts',(17.3250812297128,-21.0894161734984,-10.4409700510568));
#55351=CARTESIAN_POINT('Ctrl Pts',(17.255136354474,-21.0433106705873,-10.4451487291407));
#55352=CARTESIAN_POINT('Ctrl Pts',(17.1873530634459,-20.9936997293727,-10.4493274072247));
#55353=CARTESIAN_POINT('Ctrl Pts',(17.1221018691138,-20.940814826887,-10.4535060853086));
#55354=CARTESIAN_POINT('Ctrl Pts',(17.0556810940184,-20.8869820005319,-10.457759663194));
#55355=CARTESIAN_POINT('Ctrl Pts',(16.9918845107681,-20.8297569115571,-10.4620132410795));
#55356=CARTESIAN_POINT('Ctrl Pts',(16.9310725805954,-20.7694302518554,-10.4662668189649));
#55357=CARTESIAN_POINT('Ctrl Pts',(16.8714396083538,-20.7102731421697,-10.4704379329429));
#55358=CARTESIAN_POINT('Ctrl Pts',(16.8146769368997,-20.6481339874867,-10.4746090469208));
#55359=CARTESIAN_POINT('Ctrl Pts',(16.7610901776525,-20.5833267094255,-10.4787801608988));
#55360=CARTESIAN_POINT('Ctrl Pts',(16.70752139996,-20.5185411780723,-10.4829498752191));
#55361=CARTESIAN_POINT('Ctrl Pts',(16.6571267108674,-20.4510896556874,-10.4871195895395));
#55362=CARTESIAN_POINT('Ctrl Pts',(16.6101724826409,-20.3813203547519,-10.4912893038599));
#55363=CARTESIAN_POINT('Ctrl Pts',(16.5632199252473,-20.3115535365076,-10.4954588698039));
#55364=CARTESIAN_POINT('Ctrl Pts',(16.5197078414471,-20.2394694858256,-10.499628435748));
#55365=CARTESIAN_POINT('Ctrl Pts',(16.4798593937702,-20.1654455601081,-10.503798001692));
#55366=CARTESIAN_POINT('Ctrl Pts',(16.4386099238314,-20.0888190444807,-10.5081141644309));
#55367=CARTESIAN_POINT('Ctrl Pts',(16.4012867603007,-20.0101141681399,-10.5124303271699));
#55368=CARTESIAN_POINT('Ctrl Pts',(16.3680847835395,-19.9297756330165,-10.5167464899088));
#55369=CARTESIAN_POINT('Ctrl Pts',(16.3359643576791,-19.8520541172246,-10.5209220541005));
#55370=CARTESIAN_POINT('Ctrl Pts',(16.307700860257,-19.7728042005823,-10.5250976182921));
#55371=CARTESIAN_POINT('Ctrl Pts',(16.2834204017388,-19.6924455635533,-10.5292731824838));
#55372=CARTESIAN_POINT('Ctrl Pts',(16.257913594982,-19.6080282028025,-10.5336596444963));
#55373=CARTESIAN_POINT('Ctrl Pts',(16.236802907853,-19.522387742153,-10.5380461065089));
#55374=CARTESIAN_POINT('Ctrl Pts',(16.2201737773397,-19.4360224398369,-10.5424325685214));
#55375=CARTESIAN_POINT('Ctrl Pts',(16.2035446468265,-19.3496571375208,-10.546819030534));
#55376=CARTESIAN_POINT('Ctrl Pts',(16.1913970777482,-19.2625675787001,-10.5512054925465));
#55377=CARTESIAN_POINT('Ctrl Pts',(16.1837535357011,-19.1752553948527,-10.555591954559));
#55378=CARTESIAN_POINT('Ctrl Pts',(16.1772957565522,-19.1014881810632,-10.5592979331155));
#55379=CARTESIAN_POINT('Ctrl Pts',(16.174038011382,-19.0274367677245,-10.563003911672));
#55380=CARTESIAN_POINT('Ctrl Pts',(16.1740003306697,-18.9533011644427,-10.5667098902285));
#55381=CARTESIAN_POINT('Origin',(18.734,-18.952,1.76670989022851));
#55382=CARTESIAN_POINT('',(20.293535888361,-16.9218650751948,-9.25004024798509));
#55383=CARTESIAN_POINT('',(20.2929505583931,-16.9226084740133,-9.31680761620569));
#55384=CARTESIAN_POINT('',(20.293535888361,-16.9218650751948,1.76670989022851));
#55385=CARTESIAN_POINT('',(16.1740007840082,-18.9540035272626,-9.83329010977151));
#55386=CARTESIAN_POINT('Ctrl Pts',(20.2929505583934,-16.9226084740135,-9.31680761620571));
#55387=CARTESIAN_POINT('Ctrl Pts',(20.7827497190878,-17.3064746480848,-9.34773679031647));
#55388=CARTESIAN_POINT('Ctrl Pts',(21.6282768182897,-18.6405174171462,-9.42105789998771));
#55389=CARTESIAN_POINT('Ctrl Pts',(20.8151679945063,-21.1501879698607,-9.53677094521946));
#55390=CARTESIAN_POINT('Ctrl Pts',(18.0121685510886,-21.8917703875575,-9.66394675190086));
#55391=CARTESIAN_POINT('Ctrl Pts',(16.3483940953146,-20.372000527443,-9.76278617059769));
#55392=CARTESIAN_POINT('Ctrl Pts',(16.174290432163,-19.2372014285682,-9.81923365373404));
#55393=CARTESIAN_POINT('Ctrl Pts',(16.1763511785197,-18.9540199907297,-9.8332892013099));
#55394=CARTESIAN_POINT('Ctrl Pts',(16.1740007840082,-18.9540035272626,-9.83329010977151));
#55395=CARTESIAN_POINT('Ctrl Pts',(16.1739350379054,-18.8699966984849,-9.83745593779553));
#55396=CARTESIAN_POINT('Ctrl Pts',(16.1780086491546,-18.7859395799201,-9.84162176581955));
#55397=CARTESIAN_POINT('Ctrl Pts',(16.186209790272,-18.7022700514274,-9.84578759384357));
#55398=CARTESIAN_POINT('Ctrl Pts',(16.1944094741073,-18.6186153903909,-9.84995268163077));
#55399=CARTESIAN_POINT('Ctrl Pts',(16.2067351859308,-18.5353486407625,-9.85411776941798));
#55400=CARTESIAN_POINT('Ctrl Pts',(16.2231231591269,-18.4529033260309,-9.85828285720518));
#55401=CARTESIAN_POINT('Ctrl Pts',(16.2395131466374,-18.3704478776005,-9.86244845694076));
#55402=CARTESIAN_POINT('Ctrl Pts',(16.2599662961797,-18.2888145159801,-9.86661405667633));
#55403=CARTESIAN_POINT('Ctrl Pts',(16.284367851052,-18.2084259721855,-9.87077965641191));
#55404=CARTESIAN_POINT('Ctrl Pts',(16.308796991805,-18.127946549396,-9.87494996534484));
#55405=CARTESIAN_POINT('Ctrl Pts',(16.3371833166001,-18.0487151959129,-9.87912027427777));
#55406=CARTESIAN_POINT('Ctrl Pts',(16.3693624790262,-17.971138442795,-9.8832905832107));
#55407=CARTESIAN_POINT('Ctrl Pts',(16.4015603628991,-17.8935165564619,-9.88746331837885));
#55408=CARTESIAN_POINT('Ctrl Pts',(16.4375552801455,-17.8175516031283,-9.89163605354699));
#55409=CARTESIAN_POINT('Ctrl Pts',(16.4771361744291,-17.7436268486807,-9.89580878871514));
#55410=CARTESIAN_POINT('Ctrl Pts',(16.5167895617088,-17.6695666999467,-9.89998916630976));
#55411=CARTESIAN_POINT('Ctrl Pts',(16.5600418069661,-17.5975546086437,-9.90416954390437));
#55412=CARTESIAN_POINT('Ctrl Pts',(16.606637749578,-17.5279459787355,-9.90834992149899));
#55413=CARTESIAN_POINT('Ctrl Pts',(16.6436006876738,-17.4727278774588,-9.91166606942058));
#55414=CARTESIAN_POINT('Ctrl Pts',(16.6826668124626,-17.4190216712155,-9.91498221734216));
#55415=CARTESIAN_POINT('Ctrl Pts',(16.7236914224215,-17.3669891410737,-9.91829836526375));
#55416=CARTESIAN_POINT('Ctrl Pts',(16.7754602209958,-17.3013294900759,-9.9224829996568));
#55417=CARTESIAN_POINT('Ctrl Pts',(16.8305455538228,-17.2380865845811,-9.92666763404985));
#55418=CARTESIAN_POINT('Ctrl Pts',(16.8886933634202,-17.1776146368405,-9.93085226844289));
#55419=CARTESIAN_POINT('Ctrl Pts',(16.9467584068079,-17.1172287634326,-9.93503094652683));
#55420=CARTESIAN_POINT('Ctrl Pts',(17.0078769523774,-17.0596063422906,-9.93920962461077));
#55421=CARTESIAN_POINT('Ctrl Pts',(17.0717539579496,-17.0050695709174,-9.94338830269471));
#55422=CARTESIAN_POINT('Ctrl Pts',(17.1367759129392,-16.9495552671121,-9.94764188058015));
#55423=CARTESIAN_POINT('Ctrl Pts',(17.2046558928938,-16.897238700291,-9.95189545846559));
#55424=CARTESIAN_POINT('Ctrl Pts',(17.2750424589415,-16.8484214078413,-9.95614903635103));
#55425=CARTESIAN_POINT('Ctrl Pts',(17.3440644440582,-16.8005505338648,-9.96032015032898));
#55426=CARTESIAN_POINT('Ctrl Pts',(17.4154962970279,-16.7560447387742,-9.96449126430693));
#55427=CARTESIAN_POINT('Ctrl Pts',(17.4889737195061,-16.7151473984906,-9.96866237828488));
#55428=CARTESIAN_POINT('Ctrl Pts',(17.5624264859256,-16.6742637817044,-9.97283209260526));
#55429=CARTESIAN_POINT('Ctrl Pts',(17.6379230570026,-16.6369864384996,-9.97700180692564));
#55430=CARTESIAN_POINT('Ctrl Pts',(17.7150725574695,-16.6035139202332,-9.98117152124602));
#55431=CARTESIAN_POINT('Ctrl Pts',(17.7922193126262,-16.5700425930627,-9.98534108719006));
#55432=CARTESIAN_POINT('Ctrl Pts',(17.8710184578639,-16.5403760039564,-9.98951065313411));
#55433=CARTESIAN_POINT('Ctrl Pts',(17.9510583236146,-16.5146649119625,-9.99368021907816));
#55434=CARTESIAN_POINT('Ctrl Pts',(18.0339122923051,-16.4880498496922,-9.99799638181708));
#55435=CARTESIAN_POINT('Ctrl Pts',(18.1180953501449,-16.4656737716515,-10.002312544556));
#55436=CARTESIAN_POINT('Ctrl Pts',(18.2031347548814,-16.4476473707712,-10.0066287072949));
#55437=CARTESIAN_POINT('Ctrl Pts',(18.2854040099531,-16.4302081780035,-10.0108042714866));
#55438=CARTESIAN_POINT('Ctrl Pts',(18.3684742051326,-16.4168396609884,-10.0149798356783));
#55439=CARTESIAN_POINT('Ctrl Pts',(18.4519097174451,-16.4075894449818,-10.01915539987));
#55440=CARTESIAN_POINT('Ctrl Pts',(18.5395593591353,-16.397872022555,-10.0235418618825));
#55441=CARTESIAN_POINT('Ctrl Pts',(18.6276116092813,-16.3926998996315,-10.027928323895));
#55442=CARTESIAN_POINT('Ctrl Pts',(18.7155609817199,-16.3920664066025,-10.0323147859076));
#55443=CARTESIAN_POINT('Ctrl Pts',(18.8035103541586,-16.3914329135735,-10.0367012479201));
#55444=CARTESIAN_POINT('Ctrl Pts',(18.8913562726232,-16.395337948682,-10.0410877099327));
#55445=CARTESIAN_POINT('Ctrl Pts',(18.9786013944251,-16.403712308658,-10.0454741719452));
#55446=CARTESIAN_POINT('Ctrl Pts',(19.0618259169023,-16.4117007450961,-10.0496584884871));
#55447=CARTESIAN_POINT('Ctrl Pts',(19.1448135519499,-16.4237853774933,-10.0538428050291));
#55448=CARTESIAN_POINT('Ctrl Pts',(19.2271290458148,-16.4399443190539,-10.058027121571));
#55449=CARTESIAN_POINT('Ctrl Pts',(19.3093328037822,-16.4560813263011,-10.0622057582786));
#55450=CARTESIAN_POINT('Ctrl Pts',(19.3908657848188,-16.476281573038,-10.0663843949863));
#55451=CARTESIAN_POINT('Ctrl Pts',(19.4712973833537,-16.5004713812603,-10.0705630316939));
#55452=CARTESIAN_POINT('Ctrl Pts',(19.5516353626652,-16.5246330334953,-10.0747368046325));
#55453=CARTESIAN_POINT('Ctrl Pts',(19.6308740694797,-16.5527748851346,-10.078910577571));
#55454=CARTESIAN_POINT('Ctrl Pts',(19.7085941104905,-16.5847724402168,-10.0830843505096));
#55455=CARTESIAN_POINT('Ctrl Pts',(19.7862608039805,-16.6167480319776,-10.0872552585443));
#55456=CARTESIAN_POINT('Ctrl Pts',(19.8624104781156,-16.6525738957064,-10.0914261665791));
#55457=CARTESIAN_POINT('Ctrl Pts',(19.9366409846827,-16.6920764035124,-10.0955970746139));
#55458=CARTESIAN_POINT('Ctrl Pts',(20.0108540887567,-16.7315696504074,-10.099767004827));
#55459=CARTESIAN_POINT('Ctrl Pts',(20.0831485098601,-16.7747376197254,-10.1039369350401));
#55460=CARTESIAN_POINT('Ctrl Pts',(20.153145166604,-16.8213599562328,-10.1081068652532));
#55461=CARTESIAN_POINT('Ctrl Pts',(20.2010560885864,-16.8532717536092,-10.1109610758742));
#55462=CARTESIAN_POINT('Ctrl Pts',(20.2478909735988,-16.8868009610696,-10.1138152864951));
#55463=CARTESIAN_POINT('Ctrl Pts',(20.293535888361,-16.9218650751947,-10.1166694971161));
#55464=CARTESIAN_POINT('',(16.1740010233873,-18.9497109517325,-9.7667098901893));
#55465=CARTESIAN_POINT('Ctrl Pts',(16.174001023388,-18.9497109509451,-9.76670989022852));
#55466=CARTESIAN_POINT('Ctrl Pts',(16.1741079389015,-18.8301400729777,-9.7726651119283));
#55467=CARTESIAN_POINT('Ctrl Pts',(16.18259555166,-18.7109297707787,-9.77862033362807));
#55468=CARTESIAN_POINT('Ctrl Pts',(16.1992930219765,-18.5930285031387,-9.78457555532785));
#55469=CARTESIAN_POINT('Ctrl Pts',(16.2067339930636,-18.5404876147875,-9.78722940837539));
#55470=CARTESIAN_POINT('Ctrl Pts',(16.2158047738385,-18.4882062515533,-9.78988326142292));
#55471=CARTESIAN_POINT('Ctrl Pts',(16.2264874578014,-18.4362666864388,-9.79253711447045));
#55472=CARTESIAN_POINT('Ctrl Pts',(16.2433320704913,-18.3543676186888,-9.7967217488635));
#55473=CARTESIAN_POINT('Ctrl Pts',(16.2642246666771,-18.2731422629635,-9.80090638325655));
#55474=CARTESIAN_POINT('Ctrl Pts',(16.2890969179466,-18.193021133782,-9.80509101764959));
#55475=CARTESIAN_POINT('Ctrl Pts',(16.3139337666449,-18.1130140471109,-9.80926969573354));
#55476=CARTESIAN_POINT('Ctrl Pts',(16.3427388836329,-18.0341085006258,-9.81344837381748));
#55477=CARTESIAN_POINT('Ctrl Pts',(16.3753929533287,-17.9567247619916,-9.81762705190143));
#55478=CARTESIAN_POINT('Ctrl Pts',(16.4086323237558,-17.8779539754572,-9.82188062978686));
#55479=CARTESIAN_POINT('Ctrl Pts',(16.4458598919279,-17.8007605624573,-9.8261342076723));
#55480=CARTESIAN_POINT('Ctrl Pts',(16.4868966678982,-17.7255716022299,-9.83038778555773));
#55481=CARTESIAN_POINT('Ctrl Pts',(16.5271378658896,-17.6518403267158,-9.83455889953568));
#55482=CARTESIAN_POINT('Ctrl Pts',(16.5710416613175,-17.5800368994831,-9.83873001351364));
#55483=CARTESIAN_POINT('Ctrl Pts',(16.618391498167,-17.5105421730166,-9.8429011274916));
#55484=CARTESIAN_POINT('Ctrl Pts',(16.6657254463214,-17.4410707661768,-9.84707084181197));
#55485=CARTESIAN_POINT('Ctrl Pts',(16.7165028805482,-17.3739069013823,-9.85124055613234));
#55486=CARTESIAN_POINT('Ctrl Pts',(16.7704633948898,-17.3094032751791,-9.85541027045272));
#55487=CARTESIAN_POINT('Ctrl Pts',(16.8244219890848,-17.2449019442917,-9.85957983639676));
#55488=CARTESIAN_POINT('Ctrl Pts',(16.8815631423607,-17.1830610160833,-9.86374940234081));
#55489=CARTESIAN_POINT('Ctrl Pts',(16.9415864376593,-17.1241997862083,-9.86791896828485));
#55490=CARTESIAN_POINT('Ctrl Pts',(17.0037200779738,-17.0632690681041,-9.87223513102377));
#55491=CARTESIAN_POINT('Ctrl Pts',(17.0689419268744,-17.0055318485509,-9.87655129376269));
#55492=CARTESIAN_POINT('Ctrl Pts',(17.1368790142893,-16.9512989836053,-9.88086745650161));
#55493=CARTESIAN_POINT('Ctrl Pts',(17.2026030582275,-16.8988327485311,-9.88504302069329));
#55494=CARTESIAN_POINT('Ctrl Pts',(17.2708677497022,-16.8496463025101,-9.88921858488496));
#55495=CARTESIAN_POINT('Ctrl Pts',(17.3413050297814,-16.8039774861683,-9.89339414907664));
#55496=CARTESIAN_POINT('Ctrl Pts',(17.4152999294287,-16.7560020464804,-9.89778061108918));
#55497=CARTESIAN_POINT('Ctrl Pts',(17.4916921547951,-16.7119092180967,-9.90216707310172));
#55498=CARTESIAN_POINT('Ctrl Pts',(17.5700268579948,-16.6719196231952,-9.90655353511426));
#55499=CARTESIAN_POINT('Ctrl Pts',(17.6483615611944,-16.6319300282936,-9.91093999712679));
#55500=CARTESIAN_POINT('Ctrl Pts',(17.7286381814853,-16.5960438342244,-9.91532645913933));
#55501=CARTESIAN_POINT('Ctrl Pts',(17.8103811197834,-16.5644221134993,-9.91971292115187));
#55502=CARTESIAN_POINT('Ctrl Pts',(17.8883629443183,-16.5342553550193,-9.92389755554492));
#55503=CARTESIAN_POINT('Ctrl Pts',(17.967969380348,-16.5078569775931,-9.92808218993797));
#55504=CARTESIAN_POINT('Ctrl Pts',(18.0488014484187,-16.4854025571831,-9.93226682433102));
#55505=CARTESIAN_POINT('Ctrl Pts',(18.1295184620454,-16.4629800978612,-9.93644550241496));
#55506=CARTESIAN_POINT('Ctrl Pts',(18.2114572030593,-16.4444905669892,-9.9406241804989));
#55507=CARTESIAN_POINT('Ctrl Pts',(18.2941997096014,-16.4300611219609,-9.94480285858285));
#55508=CARTESIAN_POINT('Ctrl Pts',(18.3784253161073,-16.4153730395006,-9.94905643646828));
#55509=CARTESIAN_POINT('Ctrl Pts',(18.4634833368927,-16.404892202575,-9.95331001435371));
#55510=CARTESIAN_POINT('Ctrl Pts',(18.5489177820416,-16.3986992788558,-9.95756359223915));
#55511=CARTESIAN_POINT('Ctrl Pts',(18.6326959137598,-16.3926264170474,-9.9617347062171));
#55512=CARTESIAN_POINT('Ctrl Pts',(18.7168355246874,-16.3906767277746,-9.96590582019505));
#55513=CARTESIAN_POINT('Ctrl Pts',(18.8008991604927,-16.3928742699263,-9.97007693417301));
#55514=CARTESIAN_POINT('Ctrl Pts',(18.8849345879332,-16.3950710746715,-9.97424664849338));
#55515=CARTESIAN_POINT('Ctrl Pts',(18.96889363139,-16.4014123350032,-9.97841636281375));
#55516=CARTESIAN_POINT('Ctrl Pts',(19.0523387760777,-16.4118699986722,-9.98258607713412));
#55517=CARTESIAN_POINT('Ctrl Pts',(19.1357809514291,-16.4223272902127,-9.98675564307817));
#55518=CARTESIAN_POINT('Ctrl Pts',(19.2187088080139,-16.4369006358009,-9.99092520902221));
#55519=CARTESIAN_POINT('Ctrl Pts',(19.3006912586604,-16.4555102609148,-9.99509477496626));
#55520=CARTESIAN_POINT('Ctrl Pts',(19.3855561111354,-16.4747741774902,-9.99941093770518));
#55521=CARTESIAN_POINT('Ctrl Pts',(19.4694073254463,-16.498363368963,-10.0037271004441));
#55522=CARTESIAN_POINT('Ctrl Pts',(19.5517816392175,-16.5261324870145,-10.008043263183));
#55523=CARTESIAN_POINT('Ctrl Pts',(19.6314726183819,-16.5529970289662,-10.0122188273747));
#55524=CARTESIAN_POINT('Ctrl Pts',(19.7097810183148,-16.5837731410383,-10.0163943915664));
#55525=CARTESIAN_POINT('Ctrl Pts',(19.7863076293696,-16.6182800825355,-10.0205699557581));
#55526=CARTESIAN_POINT('Ctrl Pts',(19.866699417624,-16.6545298876152,-10.0249564177706));
#55527=CARTESIAN_POINT('Ctrl Pts',(19.9451241711511,-16.6948970480992,-10.0293428797831));
#55528=CARTESIAN_POINT('Ctrl Pts',(20.0211501810795,-16.739118527497,-10.0337293417957));
#55529=CARTESIAN_POINT('Ctrl Pts',(20.097176191008,-16.7833400068949,-10.0381158038082));
#55530=CARTESIAN_POINT('Ctrl Pts',(20.1708030131039,-16.8314154242948,-10.0425022658208));
#55531=CARTESIAN_POINT('Ctrl Pts',(20.2416377781113,-16.8830320616279,-10.0468887278333));
#55532=CARTESIAN_POINT('Ctrl Pts',(20.2590918819294,-16.8957507054557,-10.0479695779407));
#55533=CARTESIAN_POINT('Ctrl Pts',(20.2763933942624,-16.9086963274252,-10.049050428048));
#55534=CARTESIAN_POINT('Ctrl Pts',(20.293535888361,-16.9218650751948,-10.0501312781553));
#55535=CARTESIAN_POINT('Ctrl Pts',(20.293535888361,-16.9218650751948,-9.2500402479851));
#55536=CARTESIAN_POINT('Ctrl Pts',(20.3602016707525,-16.9730772773468,-9.25421688807687));
#55537=CARTESIAN_POINT('Ctrl Pts',(20.4242843944649,-17.0275322155205,-9.25839352816864));
#55538=CARTESIAN_POINT('Ctrl Pts',(20.4854677358751,-17.0849272188293,-9.26257016826041));
#55539=CARTESIAN_POINT('Ctrl Pts',(20.5467562454808,-17.1424208785499,-9.26675398758907));
#55540=CARTESIAN_POINT('Ctrl Pts',(20.6051351000148,-17.2028643650392,-9.27093780691774));
#55541=CARTESIAN_POINT('Ctrl Pts',(20.660326284079,-17.2659196201644,-9.2751216262464));
#55542=CARTESIAN_POINT('Ctrl Pts',(20.6986357799563,-17.3096877522896,-9.2780257134125));
#55543=CARTESIAN_POINT('Ctrl Pts',(20.735410269639,-17.3547135411918,-9.2809298005786));
#55544=CARTESIAN_POINT('Ctrl Pts',(20.7705691100608,-17.4008758076974,-9.2838338877447));
#55545=CARTESIAN_POINT('Ctrl Pts',(20.8212311199914,-17.4673931665203,-9.28801852213775));
#55546=CARTESIAN_POINT('Ctrl Pts',(20.8687251499199,-17.5365189656784,-9.2922031565308));
#55547=CARTESIAN_POINT('Ctrl Pts',(20.9127716012343,-17.6079187860643,-9.29638779092385));
#55548=CARTESIAN_POINT('Ctrl Pts',(20.9567553578771,-17.6792169776433,-9.30056646900779));
#55549=CARTESIAN_POINT('Ctrl Pts',(20.9973010436861,-17.7527823729939,-9.30474514709174));
#55550=CARTESIAN_POINT('Ctrl Pts',(21.0341702903065,-17.8282488551323,-9.30892382517568));
#55551=CARTESIAN_POINT('Ctrl Pts',(21.0717003916751,-17.9050680197263,-9.31317740306112));
#55552=CARTESIAN_POINT('Ctrl Pts',(21.1054206649962,-17.98385671187,-9.31743098094655));
#55553=CARTESIAN_POINT('Ctrl Pts',(21.1351268232139,-18.0641993586154,-9.32168455883198));
#55554=CARTESIAN_POINT('Ctrl Pts',(21.1642570695877,-18.1429844063778,-9.32585567280993));
#55555=CARTESIAN_POINT('Ctrl Pts',(21.1895272879509,-18.223263242189,-9.33002678678789));
#55556=CARTESIAN_POINT('Ctrl Pts',(21.2107927216344,-18.3046223559168,-9.33419790076584));
#55557=CARTESIAN_POINT('Ctrl Pts',(21.2320510194963,-18.3859541688082,-9.33836761508621));
#55558=CARTESIAN_POINT('Ctrl Pts',(21.2493070853372,-18.4683650949799,-9.34253732940659));
#55559=CARTESIAN_POINT('Ctrl Pts',(21.2624662014641,-18.5514270752364,-9.34670704372696));
#55560=CARTESIAN_POINT('Ctrl Pts',(21.2756248493332,-18.6344860997912,-9.350876609671));
#55561=CARTESIAN_POINT('Ctrl Pts',(21.284686766209,-18.7181956778687,-9.35504617561505));
#55562=CARTESIAN_POINT('Ctrl Pts',(21.2896087040397,-18.8021195415124,-9.35921574155909));
#55563=CARTESIAN_POINT('Ctrl Pts',(21.2947036911327,-18.8889940646705,-9.36353190429801));
#55564=CARTESIAN_POINT('Ctrl Pts',(21.2953621283496,-18.9760976958014,-9.36784806703693));
#55565=CARTESIAN_POINT('Ctrl Pts',(21.2915948078576,-19.0629450261169,-9.37216422977585));
#55566=CARTESIAN_POINT('Ctrl Pts',(21.2879502074343,-19.1469633137822,-9.37633979396753));
#55567=CARTESIAN_POINT('Ctrl Pts',(21.2801638500694,-19.2307412775515,-9.38051535815922));
#55568=CARTESIAN_POINT('Ctrl Pts',(21.2682983360669,-19.313845193154,-9.3846909223509));
#55569=CARTESIAN_POINT('Ctrl Pts',(21.2558335231597,-19.4011464899728,-9.38907738436344));
#55570=CARTESIAN_POINT('Ctrl Pts',(21.2388667599596,-19.487703283801,-9.39346384637597));
#55571=CARTESIAN_POINT('Ctrl Pts',(21.2175306593405,-19.5730277482655,-9.39785030838851));
#55572=CARTESIAN_POINT('Ctrl Pts',(21.1961945587214,-19.6583522127299,-9.40223677040106));
#55573=CARTESIAN_POINT('Ctrl Pts',(21.1704893630394,-19.7424438151945,-9.4066232324136));
#55574=CARTESIAN_POINT('Ctrl Pts',(21.1406062076889,-19.8248382216158,-9.41100969442614));
#55575=CARTESIAN_POINT('Ctrl Pts',(21.1120980206135,-19.9034415392599,-9.41519432881918));
#55576=CARTESIAN_POINT('Ctrl Pts',(21.0796817805212,-19.9807929863463,-9.41937896321223));
#55577=CARTESIAN_POINT('Ctrl Pts',(21.0434873395327,-20.0564764499699,-9.42356359760528));
#55578=CARTESIAN_POINT('Ctrl Pts',(21.007344416851,-20.1320521875507,-9.42774227568923));
#55579=CARTESIAN_POINT('Ctrl Pts',(20.967434172056,-20.2059642460473,-9.43192095377317));
#55580=CARTESIAN_POINT('Ctrl Pts',(20.9239354273224,-20.2778140232168,-9.43609963185711));
#55581=CARTESIAN_POINT('Ctrl Pts',(20.8796569988514,-20.3509516560045,-9.44035320974255));
#55582=CARTESIAN_POINT('Ctrl Pts',(20.8316603217325,-20.4219518942303,-9.44460678762799));
#55583=CARTESIAN_POINT('Ctrl Pts',(20.7801842503405,-20.4904180230543,-9.44886036551342));
#55584=CARTESIAN_POINT('Ctrl Pts',(20.7297061430398,-20.5575568023704,-9.45303147949137));
#55585=CARTESIAN_POINT('Ctrl Pts',(20.6758826364362,-20.6222584681312,-9.45720259346932));
#55586=CARTESIAN_POINT('Ctrl Pts',(20.6189830730721,-20.6841774776944,-9.46137370744728));
#55587=CARTESIAN_POINT('Ctrl Pts',(20.562102602906,-20.746075709736,-9.46554342176765));
#55588=CARTESIAN_POINT('Ctrl Pts',(20.5021484369599,-20.8051928015664,-9.46971313608802));
#55589=CARTESIAN_POINT('Ctrl Pts',(20.4394292363847,-20.8612174102717,-9.47388285040839));
#55590=CARTESIAN_POINT('Ctrl Pts',(20.3767122676277,-20.9172400253809,-9.47805241635244));
#55591=CARTESIAN_POINT('Ctrl Pts',(20.3112308035245,-20.9701700703296,-9.48222198229648));
#55592=CARTESIAN_POINT('Ctrl Pts',(20.2433282670354,-21.0197350367801,-9.48639154824052));
#55593=CARTESIAN_POINT('Ctrl Pts',(20.1730383611302,-21.0710426463059,-9.49070771097945));
#55594=CARTESIAN_POINT('Ctrl Pts',(20.1001543913748,-21.1187438312855,-9.49502387371837));
#55595=CARTESIAN_POINT('Ctrl Pts',(20.0250903513379,-21.162584923653,-9.49934003645729));
#55596=CARTESIAN_POINT('Ctrl Pts',(19.9524715145099,-21.2049978970479,-9.50351560064897));
#55597=CARTESIAN_POINT('Ctrl Pts',(19.8778128975685,-21.2437982255353,-9.50769116484065));
#55598=CARTESIAN_POINT('Ctrl Pts',(19.8015130783443,-21.2788037793428,-9.51186672903233));
#55599=CARTESIAN_POINT('Ctrl Pts',(19.7213595366366,-21.3155773804553,-9.51625319104487));
#55600=CARTESIAN_POINT('Ctrl Pts',(19.6393951838166,-21.3481625684723,-9.52063965305741));
#55601=CARTESIAN_POINT('Ctrl Pts',(19.5561019854972,-21.3764067986709,-9.52502611506995));
#55602=CARTESIAN_POINT('Ctrl Pts',(19.4728087871779,-21.4046510288695,-9.5294125770825));
#55603=CARTESIAN_POINT('Ctrl Pts',(19.3881873224047,-21.428554216727,-9.53379903909504));
#55604=CARTESIAN_POINT('Ctrl Pts',(19.3027314805895,-21.4480257416514,-9.53818550110758));
#55605=CARTESIAN_POINT('Ctrl Pts',(19.2212075887321,-21.4666013528504,-9.54237013550063));
#55606=CARTESIAN_POINT('Ctrl Pts',(19.1386209669249,-21.4812132961356,-9.54655476989367));
#55607=CARTESIAN_POINT('Ctrl Pts',(19.0553917867601,-21.4917455225678,-9.55073940428672));
#55608=CARTESIAN_POINT('Ctrl Pts',(18.9722810730316,-21.5022627576793,-9.55491808237067));
#55609=CARTESIAN_POINT('Ctrl Pts',(18.8885300701229,-21.508711753151,-9.55909676045461));
#55610=CARTESIAN_POINT('Ctrl Pts',(18.8045707324918,-21.5110271142986,-9.56327543853855));
#55611=CARTESIAN_POINT('Ctrl Pts',(18.7191064840742,-21.5133839766308,-9.56752901642399));
#55612=CARTESIAN_POINT('Ctrl Pts',(18.6334268287621,-21.5114574491382,-9.57178259430942));
#55613=CARTESIAN_POINT('Ctrl Pts',(18.5479946282973,-21.5052336363321,-9.57603617219486));
#55614=CARTESIAN_POINT('Ctrl Pts',(18.4642186977458,-21.499130484282,-9.58020728617281));
#55615=CARTESIAN_POINT('Ctrl Pts',(18.3806811928206,-21.4888952174951,-9.58437840015076));
#55616=CARTESIAN_POINT('Ctrl Pts',(18.2978184502102,-21.4745672747467,-9.58854951412871));
#55617=CARTESIAN_POINT('Ctrl Pts',(18.2149835129934,-21.4602441398778,-9.59271922844908));
#55618=CARTESIAN_POINT('Ctrl Pts',(18.1328233413407,-21.4418311348332,-9.59688894276945));
#55619=CARTESIAN_POINT('Ctrl Pts',(18.0517667977985,-21.4194192707795,-9.60105865708982));
#55620=CARTESIAN_POINT('Ctrl Pts',(17.9707131385959,-21.3970082042361,-9.60522822303387));
#55621=CARTESIAN_POINT('Ctrl Pts',(17.8907634725904,-21.3705986850247,-9.60939778897791));
#55622=CARTESIAN_POINT('Ctrl Pts',(17.8123328245034,-21.3403319739124,-9.61356735492196));
#55623=CARTESIAN_POINT('Ctrl Pts',(17.7311446515844,-21.3090011225754,-9.61788351766088));
#55624=CARTESIAN_POINT('Ctrl Pts',(17.651584793418,-21.2735369848544,-9.6221996803998));
#55625=CARTESIAN_POINT('Ctrl Pts',(17.5740906315704,-21.2341503581117,-9.62651584313872));
#55626=CARTESIAN_POINT('Ctrl Pts',(17.499120833894,-21.1960467465924,-9.6306914073304));
#55627=CARTESIAN_POINT('Ctrl Pts',(17.4260846045835,-21.1542725466308,-9.63486697152208));
#55628=CARTESIAN_POINT('Ctrl Pts',(17.3553508285749,-21.1090643157145,-9.63904253571376));
#55629=CARTESIAN_POINT('Ctrl Pts',(17.2810444576936,-21.061572724527,-9.6434289977263));
#55630=CARTESIAN_POINT('Ctrl Pts',(17.2092797216846,-21.010291419192,-9.64781545973884));
#55631=CARTESIAN_POINT('Ctrl Pts',(17.1404457653641,-20.9555430869522,-9.65220192175138));
#55632=CARTESIAN_POINT('Ctrl Pts',(17.0716118090436,-20.9007947547124,-9.65658838376392));
#55633=CARTESIAN_POINT('Ctrl Pts',(17.0057090169082,-20.8425798367027,-9.66097484577646));
#55634=CARTESIAN_POINT('Ctrl Pts',(16.9430809195061,-20.7812645645512,-9.665361307789));
#55635=CARTESIAN_POINT('Ctrl Pts',(16.8827886985014,-20.7222362035939,-9.66958416538901));
#55636=CARTESIAN_POINT('Ctrl Pts',(16.8252872091303,-20.6600954577447,-9.67380702298902));
#55637=CARTESIAN_POINT('Ctrl Pts',(16.7709203169311,-20.5951427685755,-9.67802988058904));
#55638=CARTESIAN_POINT('Ctrl Pts',(16.7179063153622,-20.5318063918538,-9.68214765466763));
#55639=CARTESIAN_POINT('Ctrl Pts',(16.6678730797622,-20.4657967543979,-9.68626542874624));
#55640=CARTESIAN_POINT('Ctrl Pts',(16.6211045875939,-20.3974317611818,-9.69038320282483));
#55641=CARTESIAN_POINT('Ctrl Pts',(16.57438033231,-20.329131432319,-9.69449708202704));
#55642=CARTESIAN_POINT('Ctrl Pts',(16.530914960773,-20.2584805564846,-9.69861096122925));
#55643=CARTESIAN_POINT('Ctrl Pts',(16.4909521572678,-20.1858299620347,-9.70272484043146));
#55644=CARTESIAN_POINT('Ctrl Pts',(16.4510143565681,-20.11322482157,-9.70683614577718));
#55645=CARTESIAN_POINT('Ctrl Pts',(16.4145750025456,-20.0386228602468,-9.71094745112289));
#55646=CARTESIAN_POINT('Ctrl Pts',(16.3818335581792,-19.9624024099199,-9.71505875646861));
#55647=CARTESIAN_POINT('Ctrl Pts',(16.3475554603697,-19.8826047069797,-9.719363017612));
#55648=CARTESIAN_POINT('Ctrl Pts',(16.3173311789842,-19.8010333411257,-9.72366727875539));
#55649=CARTESIAN_POINT('Ctrl Pts',(16.2913340385439,-19.718148158481,-9.72797153989879));
#55650=CARTESIAN_POINT('Ctrl Pts',(16.2665001036005,-19.6389715567965,-9.73208321292913));
#55651=CARTESIAN_POINT('Ctrl Pts',(16.245523244682,-19.5585966865051,-9.73619488595948));
#55652=CARTESIAN_POINT('Ctrl Pts',(16.2285034541843,-19.4774398718271,-9.74030655898983));
#55653=CARTESIAN_POINT('Ctrl Pts',(16.2114791195104,-19.3962613887933,-9.74441932981084));
#55654=CARTESIAN_POINT('Ctrl Pts',(16.1984140354436,-19.3143010135803,-9.74853210063185));
#55655=CARTESIAN_POINT('Ctrl Pts',(16.1893567554131,-19.2319834955465,-9.75264487145287));
#55656=CARTESIAN_POINT('Ctrl Pts',(16.1802905487374,-19.1495848472745,-9.75676169572549));
#55657=CARTESIAN_POINT('Ctrl Pts',(16.1752400549859,-19.0668288268568,-9.76087851999812));
#55658=CARTESIAN_POINT('Ctrl Pts',(16.1742017924823,-18.9841424452887,-9.76499534427075));
#55659=CARTESIAN_POINT('Ctrl Pts',(16.1740576564023,-18.9726635650768,-9.76556685957694));
#55660=CARTESIAN_POINT('Ctrl Pts',(16.1739907628404,-18.9611860219109,-9.76613837488311));
#55661=CARTESIAN_POINT('Ctrl Pts',(16.1740010233873,-18.9497109517325,-9.7667098901893));
#55662=CARTESIAN_POINT('Origin',(18.734,-18.952,1.76670989022851));
#55663=CARTESIAN_POINT('',(20.293535888361,-16.9218650751948,-8.45013430445441));
#55664=CARTESIAN_POINT('',(20.293535888361,-16.9218650751948,-8.5166771521069));
#55665=CARTESIAN_POINT('',(20.293535888361,-16.9218650751948,1.76670989022851));
#55666=CARTESIAN_POINT('',(16.1736699172806,-18.9526425113319,-9.03329016588271));
#55667=CARTESIAN_POINT('Ctrl Pts',(20.293535888361,-16.9218650751948,-8.5166771521069));
#55668=CARTESIAN_POINT('Ctrl Pts',(20.3077409125195,-16.9327772784673,-8.51757293199392));
#55669=CARTESIAN_POINT('Ctrl Pts',(20.3218260021905,-16.9438344322647,-8.51846871188095));
#55670=CARTESIAN_POINT('Ctrl Pts',(20.3357880909559,-16.9550335727229,-8.51936449176797));
#55671=CARTESIAN_POINT('Ctrl Pts',(20.4010119675945,-17.0073503405056,-8.52354912616102));
#55672=CARTESIAN_POINT('Ctrl Pts',(20.4637914133142,-17.0629632902855,-8.52773376055407));
#55673=CARTESIAN_POINT('Ctrl Pts',(20.5237743555655,-17.1216154075823,-8.53191839494712));
#55674=CARTESIAN_POINT('Ctrl Pts',(20.5836719195229,-17.1801840408498,-8.53609707303107));
#55675=CARTESIAN_POINT('Ctrl Pts',(20.6407805603835,-17.2417829302056,-8.54027575111501));
#55676=CARTESIAN_POINT('Ctrl Pts',(20.6947805623985,-17.3061143459765,-8.54445442919896));
#55677=CARTESIAN_POINT('Ctrl Pts',(20.7497484756404,-17.3715988561409,-8.54870800708439));
#55678=CARTESIAN_POINT('Ctrl Pts',(20.8014948330692,-17.4399145156592,-8.55296158496982));
#55679=CARTESIAN_POINT('Ctrl Pts',(20.8497210505507,-17.5107073731346,-8.55721516285526));
#55680=CARTESIAN_POINT('Ctrl Pts',(20.8970123087006,-17.580127772927,-8.56138627683321));
#55681=CARTESIAN_POINT('Ctrl Pts',(20.9409184275292,-17.6519297794779,-8.56555739081116));
#55682=CARTESIAN_POINT('Ctrl Pts',(20.9811990900048,-17.7257470693688,-8.56972850478912));
#55683=CARTESIAN_POINT('Ctrl Pts',(21.0214662359151,-17.7995395891552,-8.57389821910949));
#55684=CARTESIAN_POINT('Ctrl Pts',(21.0581101213991,-17.8753456457564,-8.57806793342987));
#55685=CARTESIAN_POINT('Ctrl Pts',(21.0909354749526,-17.9527727150892,-8.58223764775024));
#55686=CARTESIAN_POINT('Ctrl Pts',(21.1237596604391,-18.0301970292346,-8.58640721369428));
#55687=CARTESIAN_POINT('Ctrl Pts',(21.152765405382,-18.109241817549,-8.59057677963833));
#55688=CARTESIAN_POINT('Ctrl Pts',(21.1778054030265,-18.1894941625544,-8.59474634558237));
#55689=CARTESIAN_POINT('Ctrl Pts',(21.2037257760979,-18.2725680810081,-8.59906250832129));
#55690=CARTESIAN_POINT('Ctrl Pts',(21.2253961847597,-18.3569355479855,-8.60337867106021));
#55691=CARTESIAN_POINT('Ctrl Pts',(21.2427098983461,-18.4421229109478,-8.60769483379913));
#55692=CARTESIAN_POINT('Ctrl Pts',(21.2594596195335,-18.5245353045218,-8.61187039799081));
#55693=CARTESIAN_POINT('Ctrl Pts',(21.2721321012069,-18.60771452538,-8.61604596218248));
#55694=CARTESIAN_POINT('Ctrl Pts',(21.2806833673555,-18.6912245670413,-8.62022152637416));
#55695=CARTESIAN_POINT('Ctrl Pts',(21.2896665376286,-18.7789525023806,-8.6246079883867));
#55696=CARTESIAN_POINT('Ctrl Pts',(21.2941011966021,-18.8670449731774,-8.62899445039924));
#55697=CARTESIAN_POINT('Ctrl Pts',(21.2939982462078,-18.9549965668355,-8.63338091241178));
#55698=CARTESIAN_POINT('Ctrl Pts',(21.2938952958136,-19.0429481604935,-8.63776737442432));
#55699=CARTESIAN_POINT('Ctrl Pts',(21.2892548426303,-19.1307583016183,-8.64215383643686));
#55700=CARTESIAN_POINT('Ctrl Pts',(21.2801502518719,-19.2179302444115,-8.6465402984494));
#55701=CARTESIAN_POINT('Ctrl Pts',(21.2714645768305,-19.301091276897,-8.65072493284245));
#55702=CARTESIAN_POINT('Ctrl Pts',(21.2586842102674,-19.3839810906174,-8.65490956723549));
#55703=CARTESIAN_POINT('Ctrl Pts',(21.2418346904937,-19.4661645312117,-8.65909420162854));
#55704=CARTESIAN_POINT('Ctrl Pts',(21.2250091539259,-19.5482309938506,-8.66327287971248));
#55705=CARTESIAN_POINT('Ctrl Pts',(21.2041260603601,-19.6295926336689,-8.66745155779643));
#55706=CARTESIAN_POINT('Ctrl Pts',(21.1792626972637,-19.7098194648929,-8.67163023588037));
#55707=CARTESIAN_POINT('Ctrl Pts',(21.1539536762528,-19.7914843044085,-8.6758838137658));
#55708=CARTESIAN_POINT('Ctrl Pts',(21.1245203396143,-19.8719727727559,-8.68013739165124));
#55709=CARTESIAN_POINT('Ctrl Pts',(21.0910986865303,-19.9508422207522,-8.68439096953668));
#55710=CARTESIAN_POINT('Ctrl Pts',(21.0583249774083,-20.028182630598,-8.68856208351463));
#55711=CARTESIAN_POINT('Ctrl Pts',(21.0217164021894,-20.1039657925521,-8.69273319749258));
#55712=CARTESIAN_POINT('Ctrl Pts',(20.9814509018454,-20.1777913541034,-8.69690431147053));
#55713=CARTESIAN_POINT('Ctrl Pts',(20.9411989129789,-20.2515921427745,-8.70107402579091));
#55714=CARTESIAN_POINT('Ctrl Pts',(20.897292656152,-20.3234362321085,-8.70524374011128));
#55715=CARTESIAN_POINT('Ctrl Pts',(20.849956485239,-20.3929469638315,-8.70941345443165));
#55716=CARTESIAN_POINT('Ctrl Pts',(20.80262199875,-20.4624552220643,-8.7135830203757));
#55717=CARTESIAN_POINT('Ctrl Pts',(20.7518581004867,-20.5296299080143,-8.71775258631974));
#55718=CARTESIAN_POINT('Ctrl Pts',(20.6979322543499,-20.594123655613,-8.72192215226378));
#55719=CARTESIAN_POINT('Ctrl Pts',(20.6421104419878,-20.6608849238157,-8.7262383150027));
#55720=CARTESIAN_POINT('Ctrl Pts',(20.5829005348977,-20.7247728178031,-8.73055447774162));
#55721=CARTESIAN_POINT('Ctrl Pts',(20.5206430286226,-20.7854412148401,-8.73487064048054));
#55722=CARTESIAN_POINT('Ctrl Pts',(20.4604135540661,-20.8441333452248,-8.73904620467222));
#55723=CARTESIAN_POINT('Ctrl Pts',(20.3973323666986,-20.8998122314802,-8.7432217688639));
#55724=CARTESIAN_POINT('Ctrl Pts',(20.3317422755908,-20.9522048947021,-8.74739733305558));
#55725=CARTESIAN_POINT('Ctrl Pts',(20.2628393849067,-21.0072437867916,-8.75178379506812));
#55726=CARTESIAN_POINT('Ctrl Pts',(20.1911679546946,-21.0586554168247,-8.75617025708066));
#55727=CARTESIAN_POINT('Ctrl Pts',(20.1171588579738,-21.1061753813487,-8.76055671909321));
#55728=CARTESIAN_POINT('Ctrl Pts',(20.043149761253,-21.1536953458726,-8.76494318110575));
#55729=CARTESIAN_POINT('Ctrl Pts',(19.9668035395282,-21.1973234230529,-8.76932964311829));
#55730=CARTESIAN_POINT('Ctrl Pts',(19.8885775886028,-21.2368524223451,-8.77371610513083));
#55731=CARTESIAN_POINT('Ctrl Pts',(19.8139509296381,-21.2745626337838,-8.77790073952388));
#55732=CARTESIAN_POINT('Ctrl Pts',(19.7373359438749,-21.3086830520783,-8.78208537391693));
#55733=CARTESIAN_POINT('Ctrl Pts',(19.6591123506694,-21.3389996101045,-8.78627000830997));
#55734=CARTESIAN_POINT('Ctrl Pts',(19.5810000990668,-21.3692730162627,-8.79044868639392));
#55735=CARTESIAN_POINT('Ctrl Pts',(19.5012842132702,-21.3957531518832,-8.79462736447786));
#55736=CARTESIAN_POINT('Ctrl Pts',(19.4203680775091,-21.4182722603509,-8.7988060425618));
#55737=CARTESIAN_POINT('Ctrl Pts',(19.3380015781678,-21.4411950076538,-8.80305962044724));
#55738=CARTESIAN_POINT('Ctrl Pts',(19.2543918069889,-21.4600131107992,-8.80731319833268));
#55739=CARTESIAN_POINT('Ctrl Pts',(19.1699845756622,-21.4746013259698,-8.81156677621811));
#55740=CARTESIAN_POINT('Ctrl Pts',(19.0872137432219,-21.4889067201227,-8.81573789019606));
#55741=CARTESIAN_POINT('Ctrl Pts',(19.0036765695344,-21.4991446900207,-8.81990900417402));
#55742=CARTESIAN_POINT('Ctrl Pts',(18.9198060037776,-21.5052481526401,-8.82408011815197));
#55743=CARTESIAN_POINT('Ctrl Pts',(18.8359635815991,-21.5113495671838,-8.82824983247234));
#55744=CARTESIAN_POINT('Ctrl Pts',(18.7517884479705,-21.5133191964338,-8.83241954679272));
#55745=CARTESIAN_POINT('Ctrl Pts',(18.6677187513895,-21.5111418085137,-8.83658926111309));
#55746=CARTESIAN_POINT('Ctrl Pts',(18.5836520463691,-21.5089644980744,-8.84075882705713));
#55747=CARTESIAN_POINT('Ctrl Pts',(18.4996912307932,-21.502640476632,-8.84492839300118));
#55748=CARTESIAN_POINT('Ctrl Pts',(18.4162731576902,-21.4922066163357,-8.84909795894522));
#55749=CARTESIAN_POINT('Ctrl Pts',(18.3299222080443,-21.481405914383,-8.85341412168414));
#55750=CARTESIAN_POINT('Ctrl Pts',(18.2441533999762,-21.4662010579768,-8.85773028442306));
#55751=CARTESIAN_POINT('Ctrl Pts',(18.1594420717103,-21.4466910003124,-8.86204644716198));
#55752=CARTESIAN_POINT('Ctrl Pts',(18.0774902060527,-21.4278164807242,-8.86622201135366));
#55753=CARTESIAN_POINT('Ctrl Pts',(17.996528423794,-21.404913110059,-8.87039757554534));
#55754=CARTESIAN_POINT('Ctrl Pts',(17.916971813041,-21.3781213781908,-8.87457313973702));
#55755=CARTESIAN_POINT('Ctrl Pts',(17.8333969870066,-21.3499764596372,-8.87895960174956));
#55756=CARTESIAN_POINT('Ctrl Pts',(17.7513735563979,-21.3175402693169,-8.88334606376211));
#55757=CARTESIAN_POINT('Ctrl Pts',(17.6713570660693,-21.2810319866776,-8.88773252577465));
#55758=CARTESIAN_POINT('Ctrl Pts',(17.5913405757408,-21.2445237040383,-8.89211898778719));
#55759=CARTESIAN_POINT('Ctrl Pts',(17.513331505326,-21.203943664325,-8.89650544979973));
#55760=CARTESIAN_POINT('Ctrl Pts',(17.4377516489576,-21.159564316712,-8.90089191181227));
#55761=CARTESIAN_POINT('Ctrl Pts',(17.3656493338169,-21.1172269286685,-8.90507654620532));
#55762=CARTESIAN_POINT('Ctrl Pts',(17.295489223029,-21.0712745855039,-8.90926118059836));
#55763=CARTESIAN_POINT('Ctrl Pts',(17.227656848054,-21.0219107006307,-8.91344581499141));
#55764=CARTESIAN_POINT('Ctrl Pts',(17.1599210240689,-20.9726170791376,-8.91762449307535));
#55765=CARTESIAN_POINT('Ctrl Pts',(17.0945067235341,-20.919921829671,-8.9218031711593));
#55766=CARTESIAN_POINT('Ctrl Pts',(17.0317733474473,-20.8640733310569,-8.92598184924324));
#55767=CARTESIAN_POINT('Ctrl Pts',(16.9679155206798,-20.8072237882428,-8.93023542712867));
#55768=CARTESIAN_POINT('Ctrl Pts',(16.9068360906094,-20.7471070845336,-8.93448900501411));
#55769=CARTESIAN_POINT('Ctrl Pts',(16.8488816768787,-20.6840302849062,-8.93874258289955));
#55770=CARTESIAN_POINT('Ctrl Pts',(16.7920508225469,-20.6221763521239,-8.9429136968775));
#55771=CARTESIAN_POINT('Ctrl Pts',(16.7382252223473,-20.5574764280243,-8.94708481085545));
#55772=CARTESIAN_POINT('Ctrl Pts',(16.6876956296652,-20.4902582435822,-8.9512559248334));
#55773=CARTESIAN_POINT('Ctrl Pts',(16.6371829926759,-20.423062614851,-8.95542563915378));
#55774=CARTESIAN_POINT('Ctrl Pts',(16.5899644428517,-20.3533507714291,-8.95959535347415));
#55775=CARTESIAN_POINT('Ctrl Pts',(16.546289949262,-20.2814828821387,-8.96376506779452));
#55776=CARTESIAN_POINT('Ctrl Pts',(16.5026170097982,-20.2096175502162,-8.96793463373857));
#55777=CARTESIAN_POINT('Ctrl Pts',(16.4624881140047,-20.1355967185418,-8.97210419968261));
#55778=CARTESIAN_POINT('Ctrl Pts',(16.426108718498,-20.0598076695739,-8.97627376562665));
#55779=CARTESIAN_POINT('Ctrl Pts',(16.388450268324,-19.9813539711403,-8.98058992836557));
#55780=CARTESIAN_POINT('Ctrl Pts',(16.3548101172678,-19.9010058763734,-8.98490609110449));
#55781=CARTESIAN_POINT('Ctrl Pts',(16.3253623529171,-19.8192166309839,-8.98922225384341));
#55782=CARTESIAN_POINT('Ctrl Pts',(16.2968738463928,-19.7400916616603,-8.99339781803509));
#55783=CARTESIAN_POINT('Ctrl Pts',(16.2723088794103,-19.6596184551162,-8.99757338222677));
#55784=CARTESIAN_POINT('Ctrl Pts',(16.2517740015378,-19.5782220792646,-9.00174894641845));
#55785=CARTESIAN_POINT('Ctrl Pts',(16.230201955801,-19.4927145659702,-9.00613540843099));
#55786=CARTESIAN_POINT('Ctrl Pts',(16.213077931431,-19.4061887466983,-9.01052187044353));
#55787=CARTESIAN_POINT('Ctrl Pts',(16.2004642109875,-19.3191463002578,-9.01490833245608));
#55788=CARTESIAN_POINT('Ctrl Pts',(16.1878504905441,-19.2321038538173,-9.01929479446862));
#55789=CARTESIAN_POINT('Ctrl Pts',(16.179747051756,-19.144545364966,-9.02368125648116));
#55790=CARTESIAN_POINT('Ctrl Pts',(16.1761531171477,-19.0569729673897,-9.0280677184937));
#55791=CARTESIAN_POINT('Ctrl Pts',(16.1747268399112,-19.022219269613,-9.0298085155863));
#55792=CARTESIAN_POINT('Ctrl Pts',(16.1740088273484,-18.9874363059254,-9.0315493126789));
#55793=CARTESIAN_POINT('Ctrl Pts',(16.1740000808904,-18.9526435515772,-9.0332901097715));
#55794=CARTESIAN_POINT('Ctrl Pts',(16.1699656690245,-18.9526308403706,-9.03329079541859));
#55795=CARTESIAN_POINT('Ctrl Pts',(16.1727141322405,-18.1388729144851,-9.07394170533744));
#55796=CARTESIAN_POINT('Ctrl Pts',(17.0319371704071,-16.4715241260563,-9.15698455081677));
#55797=CARTESIAN_POINT('Ctrl Pts',(19.1726622426421,-16.2273768357865,-9.25149015774581));
#55798=CARTESIAN_POINT('Ctrl Pts',(20.1114245041509,-16.7803425872416,-9.305344854756));
#55799=CARTESIAN_POINT('Ctrl Pts',(20.2929505583934,-16.9226084740135,-9.31680761620571));
#55800=CARTESIAN_POINT('',(16.174000001606,-18.9519093211995,-8.96670989026365));
#55801=CARTESIAN_POINT('Ctrl Pts',(16.174000001606,-18.9519093211995,-8.96670989026365));
#55802=CARTESIAN_POINT('Ctrl Pts',(16.1740031377284,-18.8633718327363,-8.97108917708311));
#55803=CARTESIAN_POINT('Ctrl Pts',(16.1786036643305,-18.7749281972307,-8.97546846390257));
#55804=CARTESIAN_POINT('Ctrl Pts',(16.1877467776185,-18.6870575014995,-8.97984775072203));
#55805=CARTESIAN_POINT('Ctrl Pts',(16.1969159526897,-18.5989363367042,-8.9842395203819));
#55806=CARTESIAN_POINT('Ctrl Pts',(16.2106535575188,-18.5113917635125,-8.98863129004177));
#55807=CARTESIAN_POINT('Ctrl Pts',(16.2288531973792,-18.4248951742598,-8.99302305970163));
#55808=CARTESIAN_POINT('Ctrl Pts',(16.2470794228643,-18.3382722327341,-8.99742124475989));
#55809=CARTESIAN_POINT('Ctrl Pts',(16.2697805833342,-18.2527007028955,-9.00181942981814));
#55810=CARTESIAN_POINT('Ctrl Pts',(16.2968004138022,-18.1686366251622,-9.00621761487639));
#55811=CARTESIAN_POINT('Ctrl Pts',(16.323895396912,-18.0843387325822,-9.01062803299535));
#55812=CARTESIAN_POINT('Ctrl Pts',(16.3553329301084,-18.0015570394279,-9.0150384511143));
#55813=CARTESIAN_POINT('Ctrl Pts',(16.3909082116846,-17.9207285170583,-9.01944886923326));
#55814=CARTESIAN_POINT('Ctrl Pts',(16.4178853374885,-17.8594353629383,-9.02279333761612));
#55815=CARTESIAN_POINT('Ctrl Pts',(16.4472408225495,-17.7992649146788,-9.02613780599898));
#55816=CARTESIAN_POINT('Ctrl Pts',(16.4788683829461,-17.7403971815138,-9.02948227438184));
#55817=CARTESIAN_POINT('Ctrl Pts',(16.5184411227219,-17.6667412480013,-9.03366690877489));
#55818=CARTESIAN_POINT('Ctrl Pts',(16.5616998679758,-17.5948890389389,-9.03785154316794));
#55819=CARTESIAN_POINT('Ctrl Pts',(16.6084559713663,-17.5252335221418,-9.04203617756098));
#55820=CARTESIAN_POINT('Ctrl Pts',(16.6551455232309,-17.4556771513513,-9.04621485564493));
#55821=CARTESIAN_POINT('Ctrl Pts',(16.7053222910481,-17.3883116408714,-9.05039353372887));
#55822=CARTESIAN_POINT('Ctrl Pts',(16.7587517035101,-17.3235055519856,-9.05457221181281));
#55823=CARTESIAN_POINT('Ctrl Pts',(16.8131387997914,-17.2575378605319,-9.05882578969825));
#55824=CARTESIAN_POINT('Ctrl Pts',(16.8708960667841,-17.1942226731586,-9.06307936758369));
#55825=CARTESIAN_POINT('Ctrl Pts',(16.9317298045576,-17.1339180044288,-9.06733294546913));
#55826=CARTESIAN_POINT('Ctrl Pts',(16.9913841616171,-17.0747824593773,-9.07150405944708));
#55827=CARTESIAN_POINT('Ctrl Pts',(17.053996425417,-17.0185420838703,-9.07567517342503));
#55828=CARTESIAN_POINT('Ctrl Pts',(17.1192501263854,-16.9654998500726,-9.07984628740298));
#55829=CARTESIAN_POINT('Ctrl Pts',(17.1844819308442,-16.9124754151088,-9.08401600172335));
#55830=CARTESIAN_POINT('Ctrl Pts',(17.2523530554691,-16.8626472804565,-9.08818571604372));
#55831=CARTESIAN_POINT('Ctrl Pts',(17.3225130695871,-16.8162788933773,-9.09235543036409));
#55832=CARTESIAN_POINT('Ctrl Pts',(17.3926705871107,-16.7699121562843,-9.09652499630814));
#55833=CARTESIAN_POINT('Ctrl Pts',(17.4651164479272,-16.7270051749184,-9.10069456225218));
#55834=CARTESIAN_POINT('Ctrl Pts',(17.5394714392694,-16.6877779442822,-9.10486412819622));
#55835=CARTESIAN_POINT('Ctrl Pts',(17.6164406603804,-16.6471715326089,-9.10918029093514));
#55836=CARTESIAN_POINT('Ctrl Pts',(17.6954552934391,-16.6105086923157,-9.11349645367407));
#55837=CARTESIAN_POINT('Ctrl Pts',(17.7760690203241,-16.5779805733362,-9.11781261641299));
#55838=CARTESIAN_POINT('Ctrl Pts',(17.8540567635348,-16.5465120544111,-9.12198818060466));
#55839=CARTESIAN_POINT('Ctrl Pts',(17.933540559028,-16.5189131263825,-9.12616374479634));
#55840=CARTESIAN_POINT('Ctrl Pts',(18.0140996850992,-16.4953063812095,-9.13033930898802));
#55841=CARTESIAN_POINT('Ctrl Pts',(18.0987276611172,-16.4705073154576,-9.13472577100056));
#55842=CARTESIAN_POINT('Ctrl Pts',(18.1845418843913,-16.4501144565313,-9.13911223301311));
#55843=CARTESIAN_POINT('Ctrl Pts',(18.271043398772,-16.4342090663879,-9.14349869502565));
#55844=CARTESIAN_POINT('Ctrl Pts',(18.3575449131528,-16.4183036762444,-9.14788515703819));
#55845=CARTESIAN_POINT('Ctrl Pts',(18.4447331334585,-16.406885754803,-9.15227161905073));
#55846=CARTESIAN_POINT('Ctrl Pts',(18.5321062576864,-16.3999735665917,-9.15665808106327));
#55847=CARTESIAN_POINT('Ctrl Pts',(18.6154380422939,-16.3933810933995,-9.1608416525087));
#55848=CARTESIAN_POINT('Ctrl Pts',(18.699248101493,-16.3908622168774,-9.16502522395412));
#55849=CARTESIAN_POINT('Ctrl Pts',(18.7831042309695,-16.392470985806,-9.16920879539955));
#55850=CARTESIAN_POINT('Ctrl Pts',(18.8668503855916,-16.3940776448814,-9.17338688021372));
#55851=CARTESIAN_POINT('Ctrl Pts',(18.9506420350365,-16.3998011941729,-9.17756496502789));
#55852=CARTESIAN_POINT('Ctrl Pts',(19.0340424954886,-16.4096439075336,-9.18174304984206));
#55853=CARTESIAN_POINT('Ctrl Pts',(19.1173586063387,-16.4194766661656,-9.18591690902259));
#55854=CARTESIAN_POINT('Ctrl Pts',(19.2002838596478,-16.4334202620667,-9.19009076820312));
#55855=CARTESIAN_POINT('Ctrl Pts',(19.282383581627,-16.45142497665,-9.19426462738365));
#55856=CARTESIAN_POINT('Ctrl Pts',(19.3644249023165,-16.4694168836558,-9.19843551750712));
#55857=CARTESIAN_POINT('Ctrl Pts',(19.4456414103866,-16.4914640715301,-9.20260640763059));
#55858=CARTESIAN_POINT('Ctrl Pts',(19.5256069084354,-16.5174654443781,-9.20677729775406));
#55859=CARTESIAN_POINT('Ctrl Pts',(19.6055553058994,-16.5434612568444,-9.21094729593461));
#55860=CARTESIAN_POINT('Ctrl Pts',(19.6842527850318,-16.5734094406313,-9.21511729411516));
#55861=CARTESIAN_POINT('Ctrl Pts',(19.7612877178884,-16.6071588657916,-9.2192872922957));
#55862=CARTESIAN_POINT('Ctrl Pts',(19.8383126150258,-16.6409038942485,-9.22345674723009));
#55863=CARTESIAN_POINT('Ctrl Pts',(19.9136749774788,-16.6784489895465,-9.22762620216448));
#55864=CARTESIAN_POINT('Ctrl Pts',(19.986984126806,-16.7195952925215,-9.23179565709887));
#55865=CARTESIAN_POINT('Ctrl Pts',(20.0603319682237,-16.7607633122466,-9.23596731264437));
#55866=CARTESIAN_POINT('Ctrl Pts',(20.1316240343953,-16.8055361040649,-9.24013896818987));
#55867=CARTESIAN_POINT('Ctrl Pts',(20.2004959726216,-16.8536698157143,-9.24431062373536));
#55868=CARTESIAN_POINT('Ctrl Pts',(20.2320270456839,-16.8757064770579,-9.24622049848527));
#55869=CARTESIAN_POINT('Ctrl Pts',(20.2630512663503,-16.8984469952002,-9.24813037323518));
#55870=CARTESIAN_POINT('Ctrl Pts',(20.293535888361,-16.9218650751948,-9.2500402479851));
#55871=CARTESIAN_POINT('Ctrl Pts',(20.293535888361,-16.9218650751948,-8.45013430445441));
#55872=CARTESIAN_POINT('Ctrl Pts',(20.3602160824505,-16.9730883483156,-8.45430378930826));
#55873=CARTESIAN_POINT('Ctrl Pts',(20.4243834050837,-17.0276105723033,-8.4584732741621));
#55874=CARTESIAN_POINT('Ctrl Pts',(20.4857033632667,-17.085148284646,-8.46264275901595));
#55875=CARTESIAN_POINT('Ctrl Pts',(20.5470302074154,-17.1426924582246,-8.46681271208489));
#55876=CARTESIAN_POINT('Ctrl Pts',(20.6055087176485,-17.2032524768093,-8.47098266515382));
#55877=CARTESIAN_POINT('Ctrl Pts',(20.6608405118462,-17.266507299954,-8.47515261822275));
#55878=CARTESIAN_POINT('Ctrl Pts',(20.7162314123542,-17.3298296929158,-8.47932702570247));
#55879=CARTESIAN_POINT('Ctrl Pts',(20.7684685826588,-17.3958522904954,-8.48350143318219));
#55880=CARTESIAN_POINT('Ctrl Pts',(20.8172936355307,-17.4642205714028,-8.48767584066191));
#55881=CARTESIAN_POINT('Ctrl Pts',(20.8661466876126,-17.5326280587777,-8.49185264199692));
#55882=CARTESIAN_POINT('Ctrl Pts',(20.9115834780555,-17.6033835204386,-8.49602944333194));
#55883=CARTESIAN_POINT('Ctrl Pts',(20.9533900376111,-17.6761050744858,-8.50020624466695));
#55884=CARTESIAN_POINT('Ctrl Pts',(20.9952677497756,-17.7489503968688,-8.5043901547025));
#55885=CARTESIAN_POINT('Ctrl Pts',(21.0335026842567,-17.8237680837989,-8.50857406473805));
#55886=CARTESIAN_POINT('Ctrl Pts',(21.0679278703286,-17.9001536727719,-8.5127579747736));
#55887=CARTESIAN_POINT('Ctrl Pts',(21.0899269831306,-17.9489672125086,-8.51543166573444));
#55888=CARTESIAN_POINT('Ctrl Pts',(21.1103712768816,-17.9984206443933,-8.51810535669527));
#55889=CARTESIAN_POINT('Ctrl Pts',(21.1292278697973,-18.0484052613331,-8.5207790476561));
#55890=CARTESIAN_POINT('Ctrl Pts',(21.1587406102024,-18.1266369456353,-8.52496368204915));
#55891=CARTESIAN_POINT('Ctrl Pts',(21.1844714983967,-18.2064616309202,-8.5291483164422));
#55892=CARTESIAN_POINT('Ctrl Pts',(21.2062483053235,-18.2874788815808,-8.53333295083525));
#55893=CARTESIAN_POINT('Ctrl Pts',(21.2279941156611,-18.3683808142128,-8.53751162891918));
#55894=CARTESIAN_POINT('Ctrl Pts',(21.2457969056055,-18.4504715000486,-8.54169030700312));
#55895=CARTESIAN_POINT('Ctrl Pts',(21.2595330219156,-18.5333319271619,-8.54586898508706));
#55896=CARTESIAN_POINT('Ctrl Pts',(21.2735153482386,-18.6176775678805,-8.5501225629725));
#55897=CARTESIAN_POINT('Ctrl Pts',(21.2832836065124,-18.7028203654202,-8.55437614085793));
#55898=CARTESIAN_POINT('Ctrl Pts',(21.288760950006,-18.7883036704005,-8.55862971874337));
#55899=CARTESIAN_POINT('Ctrl Pts',(21.2941321045079,-18.8721297147068,-8.56280083272132));
#55900=CARTESIAN_POINT('Ctrl Pts',(21.2953772042646,-18.9562827012369,-8.56697194669927));
#55901=CARTESIAN_POINT('Ctrl Pts',(21.2924758541409,-19.0403249895433,-8.57114306067723));
#55902=CARTESIAN_POINT('Ctrl Pts',(21.2895754775933,-19.1243390766482,-8.5753127749976));
#55903=CARTESIAN_POINT('Ctrl Pts',(21.2825314303294,-19.2082420799253,-8.57948248931797));
#55904=CARTESIAN_POINT('Ctrl Pts',(21.2713754270314,-19.2915967348151,-8.58365220363835));
#55905=CARTESIAN_POINT('Ctrl Pts',(21.2602198207119,-19.3749484235886,-8.5878217695824));
#55906=CARTESIAN_POINT('Ctrl Pts',(21.2449526111524,-19.4577513469166,-8.59199133552645));
#55907=CARTESIAN_POINT('Ctrl Pts',(21.2256571796747,-19.539575100711,-8.5961609014705));
#55908=CARTESIAN_POINT('Ctrl Pts',(21.2056833446298,-19.6242756767481,-8.60047706420942));
#55909=CARTESIAN_POINT('Ctrl Pts',(21.1813928737509,-19.7079264335901,-8.60479322694834));
#55910=CARTESIAN_POINT('Ctrl Pts',(21.1529349892685,-19.7900653421378,-8.60910938968726));
#55911=CARTESIAN_POINT('Ctrl Pts',(21.1254041173799,-19.8695285843792,-8.61328495387894));
#55912=CARTESIAN_POINT('Ctrl Pts',(21.0939733891635,-19.9475765433411,-8.61746051807061));
#55913=CARTESIAN_POINT('Ctrl Pts',(21.058826881657,-20.0238115367569,-8.62163608226229));
#55914=CARTESIAN_POINT('Ctrl Pts',(21.0219052076091,-20.1038969784586,-8.62602254427483));
#55915=CARTESIAN_POINT('Ctrl Pts',(20.98088279295,-20.1819809787842,-8.63040900628737));
#55916=CARTESIAN_POINT('Ctrl Pts',(20.9360262797509,-20.2576340464641,-8.63479546829991));
#55917=CARTESIAN_POINT('Ctrl Pts',(20.8911697665518,-20.3332871141441,-8.63918193031245));
#55918=CARTESIAN_POINT('Ctrl Pts',(20.8424795394309,-20.4065088081494,-8.64356839232499));
#55919=CARTESIAN_POINT('Ctrl Pts',(20.790271595083,-20.4769088914603,-8.64795485433753));
#55920=CARTESIAN_POINT('Ctrl Pts',(20.7404658156452,-20.5440697625802,-8.65213948873058));
#55921=CARTESIAN_POINT('Ctrl Pts',(20.6872735296056,-20.6089129557,-8.65632412312363));
#55922=CARTESIAN_POINT('Ctrl Pts',(20.6309382156177,-20.6710769052399,-8.66050875751668));
#55923=CARTESIAN_POINT('Ctrl Pts',(20.5746830879764,-20.7331523720919,-8.66468743560061));
#55924=CARTESIAN_POINT('Ctrl Pts',(20.5152941248615,-20.7925558323524,-8.66886611368455));
#55925=CARTESIAN_POINT('Ctrl Pts',(20.4530567178388,-20.8489565100058,-8.67304479176848));
#55926=CARTESIAN_POINT('Ctrl Pts',(20.3897037500243,-20.9063681292718,-8.67729836965392));
#55927=CARTESIAN_POINT('Ctrl Pts',(20.3233995043672,-20.960667870067,-8.68155194753935));
#55928=CARTESIAN_POINT('Ctrl Pts',(20.2544863550521,-21.0115439408035,-8.68580552542479));
#55929=CARTESIAN_POINT('Ctrl Pts',(20.1869092216095,-21.0614336796322,-8.68997663940274));
#55930=CARTESIAN_POINT('Ctrl Pts',(20.1168238263198,-21.1080310270074,-8.6941477533807));
#55931=CARTESIAN_POINT('Ctrl Pts',(20.0445871160411,-21.1510819473742,-8.69831886735865));
#55932=CARTESIAN_POINT('Ctrl Pts',(19.9723746454881,-21.1941184215889,-8.70248858167902));
#55933=CARTESIAN_POINT('Ctrl Pts',(19.8980126884871,-21.2336105969123,-8.7066582959994));
#55934=CARTESIAN_POINT('Ctrl Pts',(19.82188608189,-21.2693484573603,-8.71082801031978));
#55935=CARTESIAN_POINT('Ctrl Pts',(19.7457621842044,-21.3050850461018,-8.71499757626382));
#55936=CARTESIAN_POINT('Ctrl Pts',(19.6678741785634,-21.3370673908662,-8.71916714220786));
#55937=CARTESIAN_POINT('Ctrl Pts',(19.5886290994203,-21.3651326325803,-8.7233367081519));
#55938=CARTESIAN_POINT('Ctrl Pts',(19.5065978610537,-21.3941846135709,-8.72765287089082));
#55939=CARTESIAN_POINT('Ctrl Pts',(19.4231128413873,-21.4190387397286,-8.73196903362974));
#55940=CARTESIAN_POINT('Ctrl Pts',(19.3386433049389,-21.4395703957461,-8.73628519636867));
#55941=CARTESIAN_POINT('Ctrl Pts',(19.2569253547557,-21.4594332352284,-8.74046076056034));
#55942=CARTESIAN_POINT('Ctrl Pts',(19.1742865155734,-21.4752508467085,-8.74463632475203));
#55943=CARTESIAN_POINT('Ctrl Pts',(19.0911608126529,-21.4869627519759,-8.7488118889437));
#55944=CARTESIAN_POINT('Ctrl Pts',(19.0038366280904,-21.4992661977359,-8.75319835095625));
#55945=CARTESIAN_POINT('Ctrl Pts',(18.9159756858741,-21.5070382273415,-8.75758481296879));
#55946=CARTESIAN_POINT('Ctrl Pts',(18.8280834484891,-21.5102705690994,-8.76197127498134));
#55947=CARTESIAN_POINT('Ctrl Pts',(18.740191211104,-21.5135029108574,-8.76635773699389));
#55948=CARTESIAN_POINT('Ctrl Pts',(18.6522682575723,-21.5121956494501,-8.77074419900643));
#55949=CARTESIAN_POINT('Ctrl Pts',(18.5648137584889,-21.5064032601928,-8.77513066101898));
#55950=CARTESIAN_POINT('Ctrl Pts',(18.4813831705471,-21.5008773873516,-8.77931529541202));
#55951=CARTESIAN_POINT('Ctrl Pts',(18.3980683312294,-21.4912494832414,-8.78349992980507));
#55952=CARTESIAN_POINT('Ctrl Pts',(18.3153050503467,-21.4775285662876,-8.78768456419811));
#55953=CARTESIAN_POINT('Ctrl Pts',(18.2326595727504,-21.4638271793609,-8.79186324228205));
#55954=CARTESIAN_POINT('Ctrl Pts',(18.1505645441393,-21.4460444262517,-8.79604192036599));
#55955=CARTESIAN_POINT('Ctrl Pts',(18.0694525718378,-21.4242412333191,-8.80022059844993));
#55956=CARTESIAN_POINT('Ctrl Pts',(17.9868867257269,-21.4020472338228,-8.80447417633536));
#55957=CARTESIAN_POINT('Ctrl Pts',(17.9053400062238,-21.3756872759159,-8.8087277542208));
#55958=CARTESIAN_POINT('Ctrl Pts',(17.8252599013641,-21.3452804752329,-8.81298133210624));
#55959=CARTESIAN_POINT('Ctrl Pts',(17.7467323056007,-21.3154631697152,-8.81715244608419));
#55960=CARTESIAN_POINT('Ctrl Pts',(17.6696154154526,-21.2817547038764,-8.82132356006214));
#55961=CARTESIAN_POINT('Ctrl Pts',(17.5943160431837,-21.2443177089085,-8.82549467404009));
#55962=CARTESIAN_POINT('Ctrl Pts',(17.5190419383466,-21.2068932762859,-8.82966438836045));
#55963=CARTESIAN_POINT('Ctrl Pts',(17.4455845517335,-21.1657430039572,-8.83383410268082));
#55964=CARTESIAN_POINT('Ctrl Pts',(17.3743287784402,-21.1210768011442,-8.83800381700118));
#55965=CARTESIAN_POINT('Ctrl Pts',(17.3030755407331,-21.0764121877464,-8.84217338294522));
#55966=CARTESIAN_POINT('Ctrl Pts',(17.2340241499114,-21.0282321376744,-8.84634294888926));
#55967=CARTESIAN_POINT('Ctrl Pts',(17.1675318647123,-20.9767907499611,-8.85051251483329));
#55968=CARTESIAN_POINT('Ctrl Pts',(17.0987017927924,-20.9235407465156,-8.85482867757222));
#55969=CARTESIAN_POINT('Ctrl Pts',(17.0326145482177,-20.8667961238603,-8.85914484031114));
#55970=CARTESIAN_POINT('Ctrl Pts',(16.9696289167238,-20.8068840072896,-8.86346100305007));
#55971=CARTESIAN_POINT('Ctrl Pts',(16.908695035551,-20.7489235216147,-8.86763656724175));
#55972=CARTESIAN_POINT('Ctrl Pts',(16.8506640912076,-20.6879991088316,-8.87181213143344));
#55973=CARTESIAN_POINT('Ctrl Pts',(16.7958218659397,-20.6244429797905,-8.87598769562512));
#55974=CARTESIAN_POINT('Ctrl Pts',(16.7382096902485,-20.5576767817619,-8.88037415763767));
#55975=CARTESIAN_POINT('Ctrl Pts',(16.6841171816934,-20.4880064858708,-8.88476061965021));
#55976=CARTESIAN_POINT('Ctrl Pts',(16.6338248927157,-20.4158526287654,-8.88914708166276));
#55977=CARTESIAN_POINT('Ctrl Pts',(16.583532603738,-20.3436987716601,-8.89353354367531));
#55978=CARTESIAN_POINT('Ctrl Pts',(16.537040776547,-20.2690618860433,-8.89792000568785));
#55979=CARTESIAN_POINT('Ctrl Pts',(16.4945737975988,-20.192391181845,-8.9023064677004));
#55980=CARTESIAN_POINT('Ctrl Pts',(16.4520961746315,-20.115701260729,-8.90669402914565));
#55981=CARTESIAN_POINT('Ctrl Pts',(16.4134992022811,-20.0367143701648,-8.91108159059091));
#55982=CARTESIAN_POINT('Ctrl Pts',(16.3790251742675,-19.955839414531,-8.91546915203616));
#55983=CARTESIAN_POINT('Ctrl Pts',(16.3446454932948,-19.8751857940064,-8.91984470579147));
#55984=CARTESIAN_POINT('Ctrl Pts',(16.3143664333075,-19.7926547636182,-8.92422025954678));
#55985=CARTESIAN_POINT('Ctrl Pts',(16.288384114166,-19.7086788876112,-8.9285958133021));
#55986=CARTESIAN_POINT('Ctrl Pts',(16.262443998658,-19.624839415405,-8.93296425975242));
#55987=CARTESIAN_POINT('Ctrl Pts',(16.2407868563188,-19.5395601416143,-8.93733270620274));
#55988=CARTESIAN_POINT('Ctrl Pts',(16.2235607960526,-19.4532933305799,-8.94170115265305));
#55989=CARTESIAN_POINT('Ctrl Pts',(16.2063704951608,-19.3672055997965,-8.94606053069714));
#55990=CARTESIAN_POINT('Ctrl Pts',(16.193593030381,-19.2801348014828,-8.95041990874123));
#55991=CARTESIAN_POINT('Ctrl Pts',(16.1853263642748,-19.1925466660734,-8.95477928678532));
#55992=CARTESIAN_POINT('Ctrl Pts',(16.1777850503447,-19.1126438833577,-8.95875615459972));
#55993=CARTESIAN_POINT('Ctrl Pts',(16.1739971536887,-19.0323109723967,-8.96273302241411));
#55994=CARTESIAN_POINT('Ctrl Pts',(16.174000001606,-18.95190932191,-8.96670989022851));
#55995=CARTESIAN_POINT('Origin',(18.734,-18.952,1.76670989022851));
#55996=CARTESIAN_POINT('',(20.2947700633212,-16.9202870453763,-7.65021348571703));
#55997=CARTESIAN_POINT('',(20.2923705334705,-16.9234130561299,-7.71658757622639));
#55998=CARTESIAN_POINT('',(20.293535888361,-16.9218650751948,1.76670989022851));
#55999=CARTESIAN_POINT('',(16.1740010826189,-18.9496456407634,-8.23329012251336));
#56000=CARTESIAN_POINT('Ctrl Pts',(20.2923705334702,-16.9234130561297,-7.71658757622637));
#56001=CARTESIAN_POINT('Ctrl Pts',(20.5052428179242,-17.0840214782408,-7.72982826804403));
#56002=CARTESIAN_POINT('Ctrl Pts',(21.2942513355713,-17.8922292565335,-7.78546089542218));
#56003=CARTESIAN_POINT('Ctrl Pts',(21.5288884325279,-20.114707711301,-7.88348545836079));
#56004=CARTESIAN_POINT('Ctrl Pts',(19.2691669165561,-21.9314105027038,-8.01066126504223));
#56005=CARTESIAN_POINT('Ctrl Pts',(16.7471750902531,-21.0909114965219,-8.12726281551246));
#56006=CARTESIAN_POINT('Ctrl Pts',(16.1802303010149,-19.5894613347174,-8.20147243042223));
#56007=CARTESIAN_POINT('Ctrl Pts',(16.1744184492745,-18.9496462808249,-8.23329010977151));
#56008=CARTESIAN_POINT('Ctrl Pts',(16.1740010826189,-18.9496456407634,-8.23329012251336));
#56009=CARTESIAN_POINT('Ctrl Pts',(16.1741014808467,-18.8404782076363,-8.23871812867226));
#56010=CARTESIAN_POINT('Ctrl Pts',(16.1811885397045,-18.7316228555833,-8.24414613483116));
#56011=CARTESIAN_POINT('Ctrl Pts',(16.1951208364064,-18.6238345041446,-8.24957414099005));
#56012=CARTESIAN_POINT('Ctrl Pts',(16.2083299266979,-18.5216412981712,-8.25472038679507));
#56013=CARTESIAN_POINT('Ctrl Pts',(16.2276915596983,-18.4204066645004,-8.25986663260008));
#56014=CARTESIAN_POINT('Ctrl Pts',(16.253046772176,-18.32075434152,-8.2650128784051));
#56015=CARTESIAN_POINT('Ctrl Pts',(16.2736641888711,-18.2397227402536,-8.26919751279815));
#56016=CARTESIAN_POINT('Ctrl Pts',(16.2982940662941,-18.1595514977397,-8.27338214719119));
#56017=CARTESIAN_POINT('Ctrl Pts',(16.3268482220626,-18.0806675043515,-8.27756678158424));
#56018=CARTESIAN_POINT('Ctrl Pts',(16.3553617345247,-18.0018957925641,-8.28174545966817));
#56019=CARTESIAN_POINT('Ctrl Pts',(16.3877882750862,-17.9244081193638,-8.28592413775211));
#56020=CARTESIAN_POINT('Ctrl Pts',(16.4239892031397,-17.8486187792114,-8.29010281583605));
#56021=CARTESIAN_POINT('Ctrl Pts',(16.4608390068116,-17.7714709696054,-8.29435639372148));
#56022=CARTESIAN_POINT('Ctrl Pts',(16.5015997218016,-17.6960834444034,-8.29860997160692));
#56023=CARTESIAN_POINT('Ctrl Pts',(16.5460727818104,-17.6228745401938,-8.30286354949236));
#56024=CARTESIAN_POINT('Ctrl Pts',(16.5896836447688,-17.5510849334478,-8.30703466347031));
#56025=CARTESIAN_POINT('Ctrl Pts',(16.636863945312,-17.4813906391621,-8.31120577744826));
#56026=CARTESIAN_POINT('Ctrl Pts',(16.687379731032,-17.4141620778998,-8.31537689142621));
#56027=CARTESIAN_POINT('Ctrl Pts',(16.7378785656923,-17.3469560758304,-8.31954660574659));
#56028=CARTESIAN_POINT('Ctrl Pts',(16.7917103865527,-17.2822145310262,-8.32371632006696));
#56029=CARTESIAN_POINT('Ctrl Pts',(16.8485987415143,-17.220277708609,-8.32788603438733));
#56030=CARTESIAN_POINT('Ctrl Pts',(16.9054850721441,-17.1583430901697,-8.33205560033138));
#56031=CARTESIAN_POINT('Ctrl Pts',(16.9654274088045,-17.0992133339121,-8.33622516627543));
#56032=CARTESIAN_POINT('Ctrl Pts',(17.0281108772058,-17.0431934878745,-8.34039473221947));
#56033=CARTESIAN_POINT('Ctrl Pts',(17.0929982190277,-16.9852040531582,-8.34471089495839));
#56034=CARTESIAN_POINT('Ctrl Pts',(17.160822642128,-16.9305476379184,-8.34902705769731));
#56035=CARTESIAN_POINT('Ctrl Pts',(17.2311971876102,-16.8795175013831,-8.35334322043623));
#56036=CARTESIAN_POINT('Ctrl Pts',(17.2992792896755,-16.8301496661781,-8.35751878462791));
#56037=CARTESIAN_POINT('Ctrl Pts',(17.3697475047295,-16.7841757035315,-8.3616943488196));
#56038=CARTESIAN_POINT('Ctrl Pts',(17.4422231594135,-16.7418161628216,-8.36586991301128));
#56039=CARTESIAN_POINT('Ctrl Pts',(17.5183593871211,-16.6973171424108,-8.37025637502382));
#56040=CARTESIAN_POINT('Ctrl Pts',(17.5967106568092,-16.6568075367651,-8.37464283703636));
#56041=CARTESIAN_POINT('Ctrl Pts',(17.6768123961765,-16.6204866780732,-8.3790292990489));
#56042=CARTESIAN_POINT('Ctrl Pts',(17.7569141355438,-16.5841658193814,-8.38341576106144));
#56043=CARTESIAN_POINT('Ctrl Pts',(17.8387657767031,-16.5520338488593,-8.38780222307398));
#56044=CARTESIAN_POINT('Ctrl Pts',(17.921884774769,-16.524229652346,-8.39218868508653));
#56045=CARTESIAN_POINT('Ctrl Pts',(18.0011804710186,-16.4977043913048,-8.39637337892849));
#56046=CARTESIAN_POINT('Ctrl Pts',(18.0819246518065,-16.4750187798312,-8.40055807277046));
#56047=CARTESIAN_POINT('Ctrl Pts',(18.1637106209523,-16.4563297445084,-8.40474276661243));
#56048=CARTESIAN_POINT('Ctrl Pts',(18.2453798597927,-16.437667383404,-8.40892148778458));
#56049=CARTESIAN_POINT('Ctrl Pts',(18.3280874888044,-16.4229903695745,-8.41310020895672));
#56050=CARTESIAN_POINT('Ctrl Pts',(18.4114100949884,-16.4124063803072,-8.41727893012886));
#56051=CARTESIAN_POINT('Ctrl Pts',(18.4946347461072,-16.4018348337058,-8.42145273874578));
#56052=CARTESIAN_POINT('Ctrl Pts',(18.5784724833057,-16.3953468042856,-8.42562654736271));
#56053=CARTESIAN_POINT('Ctrl Pts',(18.6624895012295,-16.3929989744891,-8.42980035597963));
#56054=CARTESIAN_POINT('Ctrl Pts',(18.7464521744712,-16.3906526633381,-8.43397146485419));
#56055=CARTESIAN_POINT('Ctrl Pts',(18.8305934396788,-16.3924412477091,-8.43814257372876));
#56056=CARTESIAN_POINT('Ctrl Pts',(18.9144752300249,-16.398369507672,-8.44231368260332));
#56057=CARTESIAN_POINT('Ctrl Pts',(18.9983279261208,-16.4042957114284,-8.44648334473617));
#56058=CARTESIAN_POINT('Ctrl Pts',(19.0819208676515,-16.4143587064509,-8.45065300686901));
#56059=CARTESIAN_POINT('Ctrl Pts',(19.1648182224782,-16.4285112127888,-8.45482266900186));
#56060=CARTESIAN_POINT('Ctrl Pts',(19.2477116915594,-16.4426630557395,-8.45899213568521));
#56061=CARTESIAN_POINT('Ctrl Pts',(19.3299091855245,-16.4609039503774,-8.46316160236856));
#56062=CARTESIAN_POINT('Ctrl Pts',(19.4109835709542,-16.4831352315977,-8.46733106905191));
#56063=CARTESIAN_POINT('Ctrl Pts',(19.4921313337444,-16.5053866335099,-8.47150430936189));
#56064=CARTESIAN_POINT('Ctrl Pts',(19.5721535125707,-16.5316355155387,-8.47567754967187));
#56065=CARTESIAN_POINT('Ctrl Pts',(19.6506371967137,-16.5617330170877,-8.47985078998185));
#56066=CARTESIAN_POINT('Ctrl Pts',(19.7291549023695,-16.591843565457,-8.48402583932959));
#56067=CARTESIAN_POINT('Ctrl Pts',(19.8061323627794,-16.6258058722132,-8.48820088867733));
#56068=CARTESIAN_POINT('Ctrl Pts',(19.8811779671305,-16.6634234310973,-8.49237593802507));
#56069=CARTESIAN_POINT('Ctrl Pts',(19.9563509512674,-16.7011048407111,-8.49655807395564));
#56070=CARTESIAN_POINT('Ctrl Pts',(20.0295851250235,-16.7424536740936,-8.50074020988622));
#56071=CARTESIAN_POINT('Ctrl Pts',(20.1005148650005,-16.7872281589662,-8.50492234581679));
#56072=CARTESIAN_POINT('Ctrl Pts',(20.1669693727351,-16.8291776480275,-8.50884061458016));
#56073=CARTESIAN_POINT('Ctrl Pts',(20.231401090238,-16.8741335444452,-8.51275888334353));
#56074=CARTESIAN_POINT('Ctrl Pts',(20.293535888361,-16.9218650751948,-8.5166771521069));
#56075=CARTESIAN_POINT('',(16.1740010575059,-18.9543268925436,-8.16670989022852));
#56076=CARTESIAN_POINT('Ctrl Pts',(16.1740010575059,-18.9543268925436,-8.16670989022852));
#56077=CARTESIAN_POINT('Ctrl Pts',(16.173925195224,-18.8708647825268,-8.17086478789788));
#56078=CARTESIAN_POINT('Ctrl Pts',(16.1779353066412,-18.7872780169979,-8.17501968556725));
#56079=CARTESIAN_POINT('Ctrl Pts',(16.1860403077383,-18.7040052286649,-8.17917458323661));
#56080=CARTESIAN_POINT('Ctrl Pts',(16.1940671586084,-18.621535375116,-8.18328941845664));
#56081=CARTESIAN_POINT('Ctrl Pts',(16.2061102365111,-18.539373952273,-8.18740425367668));
#56082=CARTESIAN_POINT('Ctrl Pts',(16.2221259449782,-18.4579466307084,-8.19151908889671));
#56083=CARTESIAN_POINT('Ctrl Pts',(16.238134689091,-18.3765547174256,-8.1956321348003));
#56084=CARTESIAN_POINT('Ctrl Pts',(16.2581125446655,-18.2958967363639,-8.19974518070389));
#56085=CARTESIAN_POINT('Ctrl Pts',(16.2819644394348,-18.216390314281,-8.20385822660748));
#56086=CARTESIAN_POINT('Ctrl Pts',(16.3058135810414,-18.136893069419,-8.2079707977528));
#56087=CARTESIAN_POINT('Ctrl Pts',(16.3335357367832,-18.0585475732033,-8.21208336889813));
#56088=CARTESIAN_POINT('Ctrl Pts',(16.3649858005362,-17.9817568744182,-8.21619594004345));
#56089=CARTESIAN_POINT('Ctrl Pts',(16.3969970744395,-17.9035958852594,-8.2203818978976));
#56090=CARTESIAN_POINT('Ctrl Pts',(16.4328704281987,-17.8270462022341,-8.22456785575175));
#56091=CARTESIAN_POINT('Ctrl Pts',(16.4724022025116,-17.7525103575288,-8.2287538136059));
#56092=CARTESIAN_POINT('Ctrl Pts',(16.5112918107485,-17.6791852955861,-8.23287177349699));
#56093=CARTESIAN_POINT('Ctrl Pts',(16.553721559467,-17.6078095092637,-8.23698973338808));
#56094=CARTESIAN_POINT('Ctrl Pts',(16.5994527799561,-17.5387384653211,-8.24110769327917));
#56095=CARTESIAN_POINT('Ctrl Pts',(16.6463167081173,-17.467956614176,-8.24532765011484));
#56096=CARTESIAN_POINT('Ctrl Pts',(16.6966475137941,-17.3995956231065,-8.24954760695052));
#56097=CARTESIAN_POINT('Ctrl Pts',(16.7501447185243,-17.3340017854889,-8.25376756378619));
#56098=CARTESIAN_POINT('Ctrl Pts',(16.8036419232545,-17.2684079478714,-8.25798752062187));
#56099=CARTESIAN_POINT('Ctrl Pts',(16.8603051182412,-17.2055816046286,-8.26220747745754));
#56100=CARTESIAN_POINT('Ctrl Pts',(16.9197953580223,-17.1458268308308,-8.26642743429322));
#56101=CARTESIAN_POINT('Ctrl Pts',(16.9787876447051,-17.0865722243692,-8.27061206868627));
#56102=CARTESIAN_POINT('Ctrl Pts',(17.040795780927,-17.0301005497847,-8.27479670307932));
#56103=CARTESIAN_POINT('Ctrl Pts',(17.1055265727615,-16.9767343731087,-8.27898133747237));
#56104=CARTESIAN_POINT('Ctrl Pts',(17.170165228326,-16.9234441565798,-8.28316001555632));
#56105=CARTESIAN_POINT('Ctrl Pts',(17.2375184898921,-16.8732509480031,-8.28733869364027));
#56106=CARTESIAN_POINT('Ctrl Pts',(17.3072561423607,-16.8264407877718,-8.29151737172421));
#56107=CARTESIAN_POINT('Ctrl Pts',(17.3782437921301,-16.7787915890601,-8.29577094960965));
#56108=CARTESIAN_POINT('Ctrl Pts',(17.4517018138304,-16.7346482555832,-8.30002452749508));
#56109=CARTESIAN_POINT('Ctrl Pts',(17.5272463530814,-16.6942698045053,-8.30427810538052));
#56110=CARTESIAN_POINT('Ctrl Pts',(17.601326314026,-16.6546741684936,-8.30844921935847));
#56111=CARTESIAN_POINT('Ctrl Pts',(17.6774121876526,-16.6186989652307,-8.31262033333642));
#56112=CARTESIAN_POINT('Ctrl Pts',(17.7551140500802,-16.5865439557984,-8.31679144731437));
#56113=CARTESIAN_POINT('Ctrl Pts',(17.8327898388975,-16.5543997362901,-8.32096116163475));
#56114=CARTESIAN_POINT('Ctrl Pts',(17.912080114858,-16.5260733404924,-8.32513087595512));
#56115=CARTESIAN_POINT('Ctrl Pts',(17.9925737212262,-16.5017169401998,-8.32930059027549));
#56116=CARTESIAN_POINT('Ctrl Pts',(18.0730644632864,-16.4773614066125,-8.33347015621953));
#56117=CARTESIAN_POINT('Ctrl Pts',(18.1547580100543,-16.4569757200691,-8.33763972216357));
#56118=CARTESIAN_POINT('Ctrl Pts',(18.2372280581077,-16.4406621816752,-8.34180928810761));
#56119=CARTESIAN_POINT('Ctrl Pts',(18.3225976513131,-16.4237750793962,-8.34612545084653));
#56120=CARTESIAN_POINT('Ctrl Pts',(18.4087988479272,-16.4112519089494,-8.35044161358545));
#56121=CARTESIAN_POINT('Ctrl Pts',(18.4953492973481,-16.4031481325656,-8.35475777632437));
#56122=CARTESIAN_POINT('Ctrl Pts',(18.5790803749826,-16.3953083358451,-8.35893334051605));
#56123=CARTESIAN_POINT('Ctrl Pts',(18.6631378283657,-16.3916044048151,-8.36310890470773));
#56124=CARTESIAN_POINT('Ctrl Pts',(18.7470834485356,-16.392033433153,-8.36728446889941));
#56125=CARTESIAN_POINT('Ctrl Pts',(18.8352689624185,-16.3924841306923,-8.37167093091196));
#56126=CARTESIAN_POINT('Ctrl Pts',(18.9233304658569,-16.3974962383813,-8.3760573929245));
#56127=CARTESIAN_POINT('Ctrl Pts',(19.0107666109435,-16.4070048638422,-8.38044385493704));
#56128=CARTESIAN_POINT('Ctrl Pts',(19.0982027560302,-16.4165134893031,-8.38483031694958));
#56129=CARTESIAN_POINT('Ctrl Pts',(19.1850129820694,-16.4305184650313,-8.38921677896212));
#56130=CARTESIAN_POINT('Ctrl Pts',(19.2707112385804,-16.4488937205181,-8.39360324097467));
#56131=CARTESIAN_POINT('Ctrl Pts',(19.3524727077245,-16.4664248576225,-8.39778819867499));
#56132=CARTESIAN_POINT('Ctrl Pts',(19.433526484304,-16.4879988204599,-8.40197315637532));
#56133=CARTESIAN_POINT('Ctrl Pts',(19.5134425416023,-16.5135436595377,-8.40615811407565));
#56134=CARTESIAN_POINT('Ctrl Pts',(19.5932250321228,-16.5390458045443,-8.41033607729535));
#56135=CARTESIAN_POINT('Ctrl Pts',(19.6718731494991,-16.5685054918704,-8.41451404051504));
#56136=CARTESIAN_POINT('Ctrl Pts',(19.7489678548332,-16.6017999545453,-8.41869200373474));
#56137=CARTESIAN_POINT('Ctrl Pts',(19.8259879712294,-16.6350622049094,-8.4228659247853));
#56138=CARTESIAN_POINT('Ctrl Pts',(19.9014572393312,-16.6721516838604,-8.42703984583586));
#56139=CARTESIAN_POINT('Ctrl Pts',(19.9749733693939,-16.7128963631723,-8.43121376688642));
#56140=CARTESIAN_POINT('Ctrl Pts',(20.0484374966371,-16.7536122210786,-8.43538473544664));
#56141=CARTESIAN_POINT('Ctrl Pts',(20.1199508294567,-16.7979779202083,-8.43955570400687));
#56142=CARTESIAN_POINT('Ctrl Pts',(20.1891338986594,-16.8457746234146,-8.4437266725671));
#56143=CARTESIAN_POINT('Ctrl Pts',(20.2245612927115,-16.8702504476067,-8.44586254986287));
#56144=CARTESIAN_POINT('Ctrl Pts',(20.2593780205127,-16.8956252326461,-8.44799842715864));
#56145=CARTESIAN_POINT('Ctrl Pts',(20.293535888361,-16.9218650751948,-8.45013430445441));
#56146=CARTESIAN_POINT('Ctrl Pts',(20.2947700633212,-16.9202870453763,-7.65021348571703));
#56147=CARTESIAN_POINT('Ctrl Pts',(20.8607342530498,-17.3635946506649,-7.68605039300052));
#56148=CARTESIAN_POINT('Ctrl Pts',(21.6914150266576,-18.8744582227272,-7.76427923584449));
#56149=CARTESIAN_POINT('Ctrl Pts',(20.547911124632,-21.3754310952809,-7.88490001424893));
#56150=CARTESIAN_POINT('Ctrl Pts',(17.6781136533722,-21.788969486026,-8.01207582093036));
#56151=CARTESIAN_POINT('Ctrl Pts',(16.2739022033865,-20.1719439048314,-8.1060124462569));
#56152=CARTESIAN_POINT('Ctrl Pts',(16.1718447244466,-19.1382186602577,-8.15755713602294));
#56153=CARTESIAN_POINT('Ctrl Pts',(16.1735502429248,-18.9543273023083,-8.16670989022852));
#56154=CARTESIAN_POINT('Origin',(18.734,-18.952,1.76670989022851));
#56155=CARTESIAN_POINT('',(20.293535888361,-16.9218650751948,-6.85004462273915));
#56156=CARTESIAN_POINT('',(20.293535888361,-16.9218650751948,-6.91673142333303));
#56157=CARTESIAN_POINT('',(20.293535888361,-16.9218650751948,1.76670989022851));
#56158=CARTESIAN_POINT('',(16.1743644997381,-18.9525601738959,-7.4332900849458));
#56159=CARTESIAN_POINT('Ctrl Pts',(20.293535888361,-16.9218650751948,-6.91673142333303));
#56160=CARTESIAN_POINT('Ctrl Pts',(20.3602014303377,-16.9730770926618,-6.9209011201467));
#56161=CARTESIAN_POINT('Ctrl Pts',(20.4243665537901,-17.0275953336019,-6.92507081696036));
#56162=CARTESIAN_POINT('Ctrl Pts',(20.4856940849898,-17.0851395787013,-6.92924051377403));
#56163=CARTESIAN_POINT('Ctrl Pts',(20.5470198579879,-17.1426821740623,-6.93341009104649));
#56164=CARTESIAN_POINT('Ctrl Pts',(20.6055078656427,-17.2032502856324,-6.93757966831895));
#56165=CARTESIAN_POINT('Ctrl Pts',(20.6608565812866,-17.2665256705744,-6.94174924559141));
#56166=CARTESIAN_POINT('Ctrl Pts',(20.7178321198183,-17.3316608609927,-6.94604137609135));
#56167=CARTESIAN_POINT('Ctrl Pts',(20.7714805826835,-17.3996645851212,-6.9503335065913));
#56168=CARTESIAN_POINT('Ctrl Pts',(20.8215177102066,-17.4701532435594,-6.95462563709125));
#56169=CARTESIAN_POINT('Ctrl Pts',(20.8701964154299,-17.5387282556663,-6.95880124360044));
#56170=CARTESIAN_POINT('Ctrl Pts',(20.9154571739033,-17.6096545653463,-6.96297685010962));
#56171=CARTESIAN_POINT('Ctrl Pts',(20.9570834061099,-17.682551234008,-6.9671524566188));
#56172=CARTESIAN_POINT('Ctrl Pts',(21.0004520635259,-17.7584992716362,-6.97150284911413));
#56173=CARTESIAN_POINT('Ctrl Pts',(21.0398749862283,-17.836585743878,-6.97585324160946));
#56174=CARTESIAN_POINT('Ctrl Pts',(21.0751622352272,-17.9163555685729,-6.98020363410478));
#56175=CARTESIAN_POINT('Ctrl Pts',(21.110449484226,-17.9961253932677,-6.98455402660011));
#56176=CARTESIAN_POINT('Ctrl Pts',(21.1416009292668,-18.077578024238,-6.98890441909544));
#56177=CARTESIAN_POINT('Ctrl Pts',(21.1684852750765,-18.1602415485544,-6.99325481159076));
#56178=CARTESIAN_POINT('Ctrl Pts',(21.194345276957,-18.2397554377671,-6.99743944598381));
#56179=CARTESIAN_POINT('Ctrl Pts',(21.216353744912,-18.320685570143,-7.00162408037686));
#56180=CARTESIAN_POINT('Ctrl Pts',(21.2343571694271,-18.4026239673097,-7.00580871476991));
#56181=CARTESIAN_POINT('Ctrl Pts',(21.2523349682957,-18.4844457353101,-7.00998739285385));
#56182=CARTESIAN_POINT('Ctrl Pts',(21.2663189491973,-18.5672724719894,-7.0141660709378));
#56183=CARTESIAN_POINT('Ctrl Pts',(21.2762049862094,-18.6506798909933,-7.01834474902174));
#56184=CARTESIAN_POINT('Ctrl Pts',(21.2862682233301,-18.735582328039,-7.02259832690718));
#56185=CARTESIAN_POINT('Ctrl Pts',(21.2920850111441,-18.8210860111299,-7.02685190479261));
#56186=CARTESIAN_POINT('Ctrl Pts',(21.2935997221946,-18.9067312233284,-7.03110548267805));
#56187=CARTESIAN_POINT('Ctrl Pts',(21.2950850676156,-18.9907160359656,-7.035276596656));
#56188=CARTESIAN_POINT('Ctrl Pts',(21.2924336475012,-19.0748364579016,-7.03944771063394));
#56189=CARTESIAN_POINT('Ctrl Pts',(21.2856453456188,-19.1586543737303,-7.04361882461189));
#56190=CARTESIAN_POINT('Ctrl Pts',(21.2788593216167,-19.2424441636477,-7.04778853893226));
#56191=CARTESIAN_POINT('Ctrl Pts',(21.2679392098803,-19.325931190906,-7.05195825325263));
#56192=CARTESIAN_POINT('Ctrl Pts',(21.252936930744,-19.4086801275884,-7.05612796757299));
#56193=CARTESIAN_POINT('Ctrl Pts',(21.2379351854531,-19.4914261197086,-7.06029753351703));
#56194=CARTESIAN_POINT('Ctrl Pts',(21.2188516444825,-19.5734336209715,-7.06446709946108));
#56195=CARTESIAN_POINT('Ctrl Pts',(21.1957895218785,-19.6542765480702,-7.06863666540512));
#56196=CARTESIAN_POINT('Ctrl Pts',(21.1719165634939,-19.7379618127552,-7.07295282814404));
#56197=CARTESIAN_POINT('Ctrl Pts',(21.1437801888442,-19.8203985795363,-7.07726899088296));
#56198=CARTESIAN_POINT('Ctrl Pts',(21.1115508461405,-19.901132221567,-7.08158515362188));
#56199=CARTESIAN_POINT('Ctrl Pts',(21.0803713708855,-19.9792359737001,-7.08576071781356));
#56200=CARTESIAN_POINT('Ctrl Pts',(21.0453617283798,-20.0557454470086,-7.08993628200524));
#56201=CARTESIAN_POINT('Ctrl Pts',(21.0067242058649,-20.1302719058331,-7.09411184619692));
#56202=CARTESIAN_POINT('Ctrl Pts',(20.9661351939398,-20.2085625189232,-7.09849830820946));
#56203=CARTESIAN_POINT('Ctrl Pts',(20.9215424772638,-20.2846640250238,-7.10288477022201));
#56204=CARTESIAN_POINT('Ctrl Pts',(20.8732322919594,-20.3581597352499,-7.10727123223455));
#56205=CARTESIAN_POINT('Ctrl Pts',(20.8249221066551,-20.4316554454761,-7.1116576942471));
#56206=CARTESIAN_POINT('Ctrl Pts',(20.7728948573422,-20.5025449370743,-7.11604415625964));
#56207=CARTESIAN_POINT('Ctrl Pts',(20.7174842649082,-20.5704530178111,-7.12043061827219));
#56208=CARTESIAN_POINT('Ctrl Pts',(20.6646231959703,-20.6352365470891,-7.12461525266523));
#56209=CARTESIAN_POINT('Ctrl Pts',(20.6084865283938,-20.6975481314174,-7.12879988705828));
#56210=CARTESIAN_POINT('Ctrl Pts',(20.5493342156371,-20.7570378626326,-7.13298452145133));
#56211=CARTESIAN_POINT('Ctrl Pts',(20.490266098876,-20.8164429175788,-7.13716319953527));
#56212=CARTESIAN_POINT('Ctrl Pts',(20.4281911845787,-20.8730337741353,-7.14134187761922));
#56213=CARTESIAN_POINT('Ctrl Pts',(20.3634098690378,-20.9264932207233,-7.14552055570316));
#56214=CARTESIAN_POINT('Ctrl Pts',(20.2974673949733,-20.9809108894708,-7.1497741335886));
#56215=CARTESIAN_POINT('Ctrl Pts',(20.2287208456647,-21.0320834094472,-7.15402771147404));
#56216=CARTESIAN_POINT('Ctrl Pts',(20.1575266602173,-21.0797151707056,-7.15828128935947));
#56217=CARTESIAN_POINT('Ctrl Pts',(20.0877127129788,-21.1264234973262,-7.16245240333742));
#56218=CARTESIAN_POINT('Ctrl Pts',(20.0155455870562,-21.1697268615303,-7.16662351731537));
#56219=CARTESIAN_POINT('Ctrl Pts',(19.9413936052584,-21.2093880220248,-7.17079463129332));
#56220=CARTESIAN_POINT('Ctrl Pts',(19.8672665058742,-21.2490358738339,-7.1749643456137));
#56221=CARTESIAN_POINT('Ctrl Pts',(19.7911562786917,-21.2850437324071,-7.17913405993407));
#56222=CARTESIAN_POINT('Ctrl Pts',(19.713457069089,-21.3172196197841,-7.18330377425445));
#56223=CARTESIAN_POINT('Ctrl Pts',(19.6357606243576,-21.3493943622049,-7.18747334019849));
#56224=CARTESIAN_POINT('Ctrl Pts',(19.5564757349844,-21.3777372293228,-7.19164290614254));
#56225=CARTESIAN_POINT('Ctrl Pts',(19.4760165374071,-21.402104377004,-7.19581247208659));
#56226=CARTESIAN_POINT('Ctrl Pts',(19.3927284937003,-21.4273282435376,-7.2001286348255));
#56227=CARTESIAN_POINT('Ctrl Pts',(19.3081825327892,-21.4482914634566,-7.20444479756443));
#56228=CARTESIAN_POINT('Ctrl Pts',(19.2228531842897,-21.4648912758434,-7.20876096030335));
#56229=CARTESIAN_POINT('Ctrl Pts',(19.1403034303424,-21.4809503510877,-7.21293652449503));
#56230=CARTESIAN_POINT('Ctrl Pts',(19.0570210156986,-21.4929259089214,-7.2171120886867));
#56231=CARTESIAN_POINT('Ctrl Pts',(18.9734422997763,-21.5007776256625,-7.22128765287838));
#56232=CARTESIAN_POINT('Ctrl Pts',(18.8856422216022,-21.5090259139505,-7.22567411489092));
#56233=CARTESIAN_POINT('Ctrl Pts',(18.7975157065272,-21.5127227980494,-7.23006057690346));
#56234=CARTESIAN_POINT('Ctrl Pts',(18.7095680581453,-21.5118834114501,-7.234447038916));
#56235=CARTESIAN_POINT('Ctrl Pts',(18.6216204097634,-21.5110440248507,-7.23883350092854));
#56236=CARTESIAN_POINT('Ctrl Pts',(18.5338522025563,-21.5056684789459,-7.24321996294108));
#56237=CARTESIAN_POINT('Ctrl Pts',(18.4467595506041,-21.4958342957494,-7.24760642495362));
#56238=CARTESIAN_POINT('Ctrl Pts',(18.3636741606704,-21.4864525978996,-7.25179105934667));
#56239=CARTESIAN_POINT('Ctrl Pts',(18.2808942658294,-21.4729786230522,-7.25597569373971));
#56240=CARTESIAN_POINT('Ctrl Pts',(18.1988547913486,-21.4554415522751,-7.26016032813276));
#56241=CARTESIAN_POINT('Ctrl Pts',(18.1169320899053,-21.4379294433475,-7.26433900621671));
#56242=CARTESIAN_POINT('Ctrl Pts',(18.0357481614732,-21.4163658213152,-7.26851768430065));
#56243=CARTESIAN_POINT('Ctrl Pts',(17.955732329606,-21.3908315713102,-7.2726963623846));
#56244=CARTESIAN_POINT('Ctrl Pts',(17.874282271459,-21.3648396382251,-7.27694994027003));
#56245=CARTESIAN_POINT('Ctrl Pts',(17.7940430771264,-21.3347333841335,-7.28120351815547));
#56246=CARTESIAN_POINT('Ctrl Pts',(17.7154562415196,-21.3006525098576,-7.2854570960409));
#56247=CARTESIAN_POINT('Ctrl Pts',(17.6383929650706,-21.267232359833,-7.28962821001885));
#56248=CARTESIAN_POINT('Ctrl Pts',(17.5629189921768,-21.2299905173578,-7.2937993239968));
#56249=CARTESIAN_POINT('Ctrl Pts',(17.4894331713722,-21.1891082694137,-7.29797043797475));
#56250=CARTESIAN_POINT('Ctrl Pts',(17.4159720094442,-21.1482397399027,-7.30214015229513));
#56251=CARTESIAN_POINT('Ctrl Pts',(17.3444980763221,-21.1037334544494,-7.3063098666155));
#56252=CARTESIAN_POINT('Ctrl Pts',(17.2753861385067,-21.0558169129132,-7.31047958093588));
#56253=CARTESIAN_POINT('Ctrl Pts',(17.2062766599909,-21.0079020764533,-7.31464914687992));
#56254=CARTESIAN_POINT('Ctrl Pts',(17.13952938724,-20.9565774880023,-7.31881871282395));
#56255=CARTESIAN_POINT('Ctrl Pts',(17.0754894346057,-20.9021135106643,-7.32298827876799));
#56256=CARTESIAN_POINT('Ctrl Pts',(17.0091979162385,-20.8457346470716,-7.32730444150691));
#56257=CARTESIAN_POINT('Ctrl Pts',(16.9458080406879,-20.7859918669771,-7.33162060424583));
#56258=CARTESIAN_POINT('Ctrl Pts',(16.8856630675041,-20.7232285521557,-7.33593676698476));
#56259=CARTESIAN_POINT('Ctrl Pts',(16.8274773104957,-20.6625097457132,-7.34011233117643));
#56260=CARTESIAN_POINT('Ctrl Pts',(16.7723285700599,-20.5989645570466,-7.34428789536811));
#56261=CARTESIAN_POINT('Ctrl Pts',(16.7204869451086,-20.5329380689268,-7.34846345955979));
#56262=CARTESIAN_POINT('Ctrl Pts',(16.6660269229228,-20.4635767398551,-7.35284992157233));
#56263=CARTESIAN_POINT('Ctrl Pts',(16.6152172172816,-20.3914773402461,-7.35723638358488));
#56264=CARTESIAN_POINT('Ctrl Pts',(16.5683186145658,-20.317072941928,-7.36162284559742));
#56265=CARTESIAN_POINT('Ctrl Pts',(16.52142001185,-20.2426685436098,-7.36600930760997));
#56266=CARTESIAN_POINT('Ctrl Pts',(16.4784327293519,-20.1659596899256,-7.37039576962251));
#56267=CARTESIAN_POINT('Ctrl Pts',(16.4395601204679,-20.0874054955004,-7.37478223163505));
#56268=CARTESIAN_POINT('Ctrl Pts',(16.3997963941391,-20.0070505211682,-7.37926924910123));
#56269=CARTESIAN_POINT('Ctrl Pts',(16.3642056179145,-19.9244993534859,-7.38375626656741));
#56270=CARTESIAN_POINT('Ctrl Pts',(16.333017909016,-19.8401919830611,-7.38824328403359));
#56271=CARTESIAN_POINT('Ctrl Pts',(16.3019356806124,-19.7561697500662,-7.39271512587963));
#56272=CARTESIAN_POINT('Ctrl Pts',(16.2752269677052,-19.6704034844248,-7.39718696772568));
#56273=CARTESIAN_POINT('Ctrl Pts',(16.2530742870064,-19.5833537887801,-7.40165880957172));
#56274=CARTESIAN_POINT('Ctrl Pts',(16.2309688572623,-19.4964897673338,-7.40612111312307));
#56275=CARTESIAN_POINT('Ctrl Pts',(16.2134002030054,-19.408348109083,-7.41058341667443));
#56276=CARTESIAN_POINT('Ctrl Pts',(16.2005019648758,-19.3194067310513,-7.41504572022578));
#56277=CARTESIAN_POINT('Ctrl Pts',(16.1876417930136,-19.2307278436206,-7.41949485428542));
#56278=CARTESIAN_POINT('Ctrl Pts',(16.1794246278367,-19.1412542906273,-7.42394398834506));
#56279=CARTESIAN_POINT('Ctrl Pts',(16.175933399183,-19.0514749505386,-7.4283931224047));
#56280=CARTESIAN_POINT('Ctrl Pts',(16.1746525201579,-19.0185362676236,-7.43002544244505));
#56281=CARTESIAN_POINT('Ctrl Pts',(16.1740072831437,-18.9855565464226,-7.4316577624854));
#56282=CARTESIAN_POINT('Ctrl Pts',(16.1740000613162,-18.952560302501,-7.43329008252576));
#56283=CARTESIAN_POINT('Ctrl Pts',(16.1781030393919,-18.952558854618,-7.43329010977151));
#56284=CARTESIAN_POINT('Ctrl Pts',(16.1790025482941,-18.4906083143692,-7.4561794192865));
#56285=CARTESIAN_POINT('Ctrl Pts',(16.5197425194489,-17.1718695770502,-7.52146066436197));
#56286=CARTESIAN_POINT('Ctrl Pts',(18.3750628649076,-16.0796619494175,-7.61589315318027));
#56287=CARTESIAN_POINT('Ctrl Pts',(19.8237022844342,-16.5698110446498,-7.68743633248356));
#56288=CARTESIAN_POINT('Ctrl Pts',(20.2923705334702,-16.9234130561297,-7.71658757622637));
#56289=CARTESIAN_POINT('',(16.1738764939443,-18.9508698166505,-7.36670989022851));
#56290=CARTESIAN_POINT('Ctrl Pts',(16.170378839146,-18.9508682725878,-7.36670989022851));
#56291=CARTESIAN_POINT('Ctrl Pts',(16.1700290602903,-18.8875375837258,-7.36987218932674));
#56292=CARTESIAN_POINT('Ctrl Pts',(16.2008981559486,-17.9755793377669,-7.41542642398544));
#56293=CARTESIAN_POINT('Ctrl Pts',(17.2895132774888,-16.291783852743,-7.50337259420463));
#56294=CARTESIAN_POINT('Ctrl Pts',(19.3719151115967,-16.2958825772312,-7.59471149360257));
#56295=CARTESIAN_POINT('Ctrl Pts',(20.1912479809582,-16.8392004196504,-7.64365845744004));
#56296=CARTESIAN_POINT('Ctrl Pts',(20.2947700633212,-16.9202870453763,-7.65021348571703));
#56297=CARTESIAN_POINT('Ctrl Pts',(20.293535888361,-16.9218650751948,-6.85004462273914));
#56298=CARTESIAN_POINT('Ctrl Pts',(20.3601338996604,-16.9730252160533,-6.85422899536763));
#56299=CARTESIAN_POINT('Ctrl Pts',(20.4241220221326,-17.0273968372747,-6.85841336799612));
#56300=CARTESIAN_POINT('Ctrl Pts',(20.4851928160501,-17.0846693594828,-6.8625977406246));
#56301=CARTESIAN_POINT('Ctrl Pts',(20.5090109325979,-17.1070061185362,-6.86422968068222));
#56302=CARTESIAN_POINT('Ctrl Pts',(20.5323857251923,-17.1297837513318,-6.86586162073984));
#56303=CARTESIAN_POINT('Ctrl Pts',(20.5553006227462,-17.1529824788,-6.86749356079746));
#56304=CARTESIAN_POINT('Ctrl Pts',(20.6140591953844,-17.2124688504871,-6.87167819519051));
#56305=CARTESIAN_POINT('Ctrl Pts',(20.6700096812721,-17.2749476638323,-6.87586282958355));
#56306=CARTESIAN_POINT('Ctrl Pts',(20.7228319806688,-17.3401230342644,-6.8800474639766));
#56307=CARTESIAN_POINT('Ctrl Pts',(20.7755790940605,-17.4052056356238,-6.88422614206054));
#56308=CARTESIAN_POINT('Ctrl Pts',(20.8252065780214,-17.4729768158299,-6.88840482014449));
#56309=CARTESIAN_POINT('Ctrl Pts',(20.8714311671561,-17.5431039762745,-6.89258349822843));
#56310=CARTESIAN_POINT('Ctrl Pts',(20.9184842988301,-17.6144881156706,-6.89683707611387));
#56311=CARTESIAN_POINT('Ctrl Pts',(20.9620110031542,-17.6883131849442,-6.90109065399931));
#56312=CARTESIAN_POINT('Ctrl Pts',(21.0017554861493,-17.7641931743588,-6.90534423188474));
#56313=CARTESIAN_POINT('Ctrl Pts',(21.0407294447865,-17.838602082111,-6.90951534586269));
#56314=CARTESIAN_POINT('Ctrl Pts',(21.0760663016048,-17.9149865174727,-6.91368645984064));
#56315=CARTESIAN_POINT('Ctrl Pts',(21.1075695674518,-17.9929548975847,-6.9178575738186));
#56316=CARTESIAN_POINT('Ctrl Pts',(21.1390622620736,-18.0708971146537,-6.92202728813897));
#56317=CARTESIAN_POINT('Ctrl Pts',(21.1667237483346,-18.1504217947136,-6.92619700245934));
#56318=CARTESIAN_POINT('Ctrl Pts',(21.1904053024889,-18.2311165212712,-6.93036671677971));
#56319=CARTESIAN_POINT('Ctrl Pts',(21.214086013952,-18.3118083763641,-6.93453628272375));
#56320=CARTESIAN_POINT('Ctrl Pts',(21.2337869461661,-18.3936697535163,-6.9387058486678));
#56321=CARTESIAN_POINT('Ctrl Pts',(21.2494093711531,-18.4762735076587,-6.94287541461184));
#56322=CARTESIAN_POINT('Ctrl Pts',(21.2655810613302,-18.561781507894,-6.94719157735076));
#56323=CARTESIAN_POINT('Ctrl Pts',(21.2773820094429,-18.6480845421362,-6.95150774008968));
#56324=CARTESIAN_POINT('Ctrl Pts',(21.2847607940422,-18.7346998122938,-6.9558239028286));
#56325=CARTESIAN_POINT('Ctrl Pts',(21.2918992155093,-18.8184935991363,-6.95999946702028));
#56326=CARTESIAN_POINT('Ctrl Pts',(21.2948991834511,-18.9025791196893,-6.96417503121196));
#56327=CARTESIAN_POINT('Ctrl Pts',(21.2937672733171,-18.9865182046883,-6.96835059540364));
#56328=CARTESIAN_POINT('Ctrl Pts',(21.2925781930931,-19.0746968533244,-6.97273705741618));
#56329=CARTESIAN_POINT('Ctrl Pts',(21.2868289009943,-19.1627133020808,-6.97712351942873));
#56330=CARTESIAN_POINT('Ctrl Pts',(21.2765884850301,-19.250066763985,-6.98150998144127));
#56331=CARTESIAN_POINT('Ctrl Pts',(21.2663480690658,-19.3374202258893,-6.98589644345381));
#56332=CARTESIAN_POINT('Ctrl Pts',(21.2516167014297,-19.4241101416678,-6.99028290546635));
#56333=CARTESIAN_POINT('Ctrl Pts',(21.2325245180281,-19.5096515334976,-6.9946693674789));
#56334=CARTESIAN_POINT('Ctrl Pts',(21.2143107942863,-19.5912570390866,-6.99885400187194));
#56335=CARTESIAN_POINT('Ctrl Pts',(21.1920609365757,-19.6721211400212,-7.00303863626499));
#56336=CARTESIAN_POINT('Ctrl Pts',(21.1658504730776,-19.75181452637,-7.00722327065804));
#56337=CARTESIAN_POINT('Ctrl Pts',(21.1396773169301,-19.8313944790474,-7.01140194874198));
#56338=CARTESIAN_POINT('Ctrl Pts',(21.1095548952069,-19.9098065938023,-7.01558062682592));
#56339=CARTESIAN_POINT('Ctrl Pts',(21.0756095445167,-19.9866326599466,-7.01975930490986));
#56340=CARTESIAN_POINT('Ctrl Pts',(21.0410557478115,-20.0648357781127,-7.0240128827953));
#56341=CARTESIAN_POINT('Ctrl Pts',(21.0025407271242,-20.1413949579936,-7.02826646068074));
#56342=CARTESIAN_POINT('Ctrl Pts',(20.9602505991267,-20.215886177584,-7.03252003856617));
#56343=CARTESIAN_POINT('Ctrl Pts',(20.9187803477829,-20.2889332395249,-7.03669115254412));
#56344=CARTESIAN_POINT('Ctrl Pts',(20.8736802961219,-20.3599913900462,-7.04086226652207));
#56345=CARTESIAN_POINT('Ctrl Pts',(20.8251733475076,-20.4286834564909,-7.04503338050002));
#56346=CARTESIAN_POINT('Ctrl Pts',(20.7766826758684,-20.4973524726493,-7.0492030948204));
#56347=CARTESIAN_POINT('Ctrl Pts',(20.724787642863,-20.5636566060812,-7.05337280914077));
#56348=CARTESIAN_POINT('Ctrl Pts',(20.669754524153,-20.6272475704269,-7.05754252346114));
#56349=CARTESIAN_POINT('Ctrl Pts',(20.6147233637574,-20.6908362719332,-7.06171208940519));
#56350=CARTESIAN_POINT('Ctrl Pts',(20.556554641366,-20.7517116490139,-7.06588165534923));
#56351=CARTESIAN_POINT('Ctrl Pts',(20.4955540788024,-20.8095594815387,-7.07005122129327));
#56352=CARTESIAN_POINT('Ctrl Pts',(20.4324088117115,-20.8694411724922,-7.07436738403219));
#56353=CARTESIAN_POINT('Ctrl Pts',(20.3662292470559,-20.9260780978832,-7.07868354677112));
#56354=CARTESIAN_POINT('Ctrl Pts',(20.2973935081709,-20.9791656909609,-7.08299970951004));
#56355=CARTESIAN_POINT('Ctrl Pts',(20.2308000862399,-21.030523961278,-7.08717527370171));
#56356=CARTESIAN_POINT('Ctrl Pts',(20.1617212960249,-21.0785603570292,-7.09135083789339));
#56357=CARTESIAN_POINT('Ctrl Pts',(20.0905291277018,-21.1230432344144,-7.09552640208507));
#56358=CARTESIAN_POINT('Ctrl Pts',(20.0157412122,-21.1697728361884,-7.09991286409761));
#56359=CARTESIAN_POINT('Ctrl Pts',(19.9386213249318,-21.2125802257264,-7.10429932611016));
#56360=CARTESIAN_POINT('Ctrl Pts',(19.8596279445188,-21.2512524286207,-7.1086857881227));
#56361=CARTESIAN_POINT('Ctrl Pts',(19.7806345641058,-21.2899246315151,-7.11307225013524));
#56362=CARTESIAN_POINT('Ctrl Pts',(19.6997682540138,-21.3244614898292,-7.11745871214778));
#56363=CARTESIAN_POINT('Ctrl Pts',(19.6175072439402,-21.3547099179687,-7.12184517416032));
#56364=CARTESIAN_POINT('Ctrl Pts',(19.5390311848803,-21.3835665710906,-7.12602980855337));
#56365=CARTESIAN_POINT('Ctrl Pts',(19.4589938470389,-21.4086281659991,-7.13021444294642));
#56366=CARTESIAN_POINT('Ctrl Pts',(19.3777970941006,-21.429725832619,-7.13439907733946));
#56367=CARTESIAN_POINT('Ctrl Pts',(19.29671591469,-21.4507934693218,-7.13857775542341));
#56368=CARTESIAN_POINT('Ctrl Pts',(19.2144790396054,-21.4679082701427,-7.14275643350735));
#56369=CARTESIAN_POINT('Ctrl Pts',(19.1315065014624,-21.4809500946628,-7.1469351115913));
#56370=CARTESIAN_POINT('Ctrl Pts',(19.0470467402045,-21.4942256845145,-7.15118868947673));
#56371=CARTESIAN_POINT('Ctrl Pts',(18.9618251354747,-21.5032806792605,-7.15544226736217));
#56372=CARTESIAN_POINT('Ctrl Pts',(18.876298964101,-21.508042058499,-7.15969584524761));
#56373=CARTESIAN_POINT('Ctrl Pts',(18.7924308844499,-21.5127111291099,-7.16386695922556));
#56374=CARTESIAN_POINT('Ctrl Pts',(18.7082704224837,-21.5132515520536,-7.16803807320351));
#56375=CARTESIAN_POINT('Ctrl Pts',(18.624255374081,-21.5096465973785,-7.17220918718146));
#56376=CARTESIAN_POINT('Ctrl Pts',(18.5402685177392,-21.5060428523808,-7.17637890150184));
#56377=CARTESIAN_POINT('Ctrl Pts',(18.4564274372809,-21.4982965120596,-7.18054861582221));
#56378=CARTESIAN_POINT('Ctrl Pts',(18.3731691163824,-21.4864429513066,-7.18471833014259));
#56379=CARTESIAN_POINT('Ctrl Pts',(18.2899137581722,-21.4745898123542,-7.18888789608663));
#56380=CARTESIAN_POINT('Ctrl Pts',(18.2072415736112,-21.4586298092437,-7.19305746203067));
#56381=CARTESIAN_POINT('Ctrl Pts',(18.1255822535273,-21.4386499242509,-7.19722702797472));
#56382=CARTESIAN_POINT('Ctrl Pts',(18.0410518924869,-21.4179675711496,-7.20154319071364));
#56383=CARTESIAN_POINT('Ctrl Pts',(17.9576074580674,-21.3929775239273,-7.20585935345255));
#56384=CARTESIAN_POINT('Ctrl Pts',(17.8757097136974,-21.363832868264,-7.21017551619147));
#56385=CARTESIAN_POINT('Ctrl Pts',(17.7964797797361,-21.3356375966935,-7.21435108038315));
#56386=CARTESIAN_POINT('Ctrl Pts',(17.7186977338733,-21.303554456016,-7.21852664457484));
#56387=CARTESIAN_POINT('Ctrl Pts',(17.6427597031132,-21.2677708467054,-7.22270220876652));
#56388=CARTESIAN_POINT('Ctrl Pts',(17.562986222945,-21.2301798923558,-7.22708867077906));
#56389=CARTESIAN_POINT('Ctrl Pts',(17.4852484504759,-21.1885050997006,-7.2314751327916));
#56390=CARTESIAN_POINT('Ctrl Pts',(17.4099736292609,-21.1430166976971,-7.23586159480414));
#56391=CARTESIAN_POINT('Ctrl Pts',(17.334698808046,-21.0975282956936,-7.24024805681668));
#56392=CARTESIAN_POINT('Ctrl Pts',(17.2618873758782,-21.0482266726393,-7.24463451882922));
#56393=CARTESIAN_POINT('Ctrl Pts',(17.1919269101811,-20.9954310816997,-7.24902098084176));
#56394=CARTESIAN_POINT('Ctrl Pts',(17.1258771580207,-20.9455867065661,-7.25316224442402));
#56395=CARTESIAN_POINT('Ctrl Pts',(17.0621112325388,-20.892434299838,-7.25730350800628));
#56396=CARTESIAN_POINT('Ctrl Pts',(17.0009846311415,-20.8362127616859,-7.26144477158854));
#56397=CARTESIAN_POINT('Ctrl Pts',(16.9399453026366,-20.7800714932715,-7.26558012252322));
#56398=CARTESIAN_POINT('Ctrl Pts',(16.8815381604268,-20.7208701082194,-7.26971547345791));
#56399=CARTESIAN_POINT('Ctrl Pts',(16.8260879518442,-20.6588894564388,-7.27385082439259));
#56400=CARTESIAN_POINT('Ctrl Pts',(16.770701311821,-20.5969798597695,-7.27798143452813));
#56401=CARTESIAN_POINT('Ctrl Pts',(16.7182651826551,-20.5322976752766,-7.28211204466367));
#56402=CARTESIAN_POINT('Ctrl Pts',(16.6690684130046,-20.4651614391824,-7.2862426547992));
#56403=CARTESIAN_POINT('Ctrl Pts',(16.6199019406792,-20.3980665482496,-7.29037072114092));
#56404=CARTESIAN_POINT('Ctrl Pts',(16.5739711466917,-20.3285209831314,-7.29449878748264));
#56405=CARTESIAN_POINT('Ctrl Pts',(16.5315246255303,-20.2568763255016,-7.29862685382436));
#56406=CARTESIAN_POINT('Ctrl Pts',(16.4890908665707,-20.185253208944,-7.30275367899921));
#56407=CARTESIAN_POINT('Ctrl Pts',(16.4501395400175,-20.1115326575802,-7.30688050417406));
#56408=CARTESIAN_POINT('Ctrl Pts',(16.4148750854128,-20.0360939214575,-7.31100732934891));
#56409=CARTESIAN_POINT('Ctrl Pts',(16.3796101195077,-19.9606540915462,-7.31513421435872));
#56410=CARTESIAN_POINT('Ctrl Pts',(16.3480323287909,-19.8834964546655,-7.31926109936854));
#56411=CARTESIAN_POINT('Ctrl Pts',(16.320298833946,-19.8050220870468,-7.32338798437836));
#56412=CARTESIAN_POINT('Ctrl Pts',(16.2925397363851,-19.7264752742868,-7.32751867920247));
#56413=CARTESIAN_POINT('Ctrl Pts',(16.2686321752694,-19.646609748954,-7.33164937402659));
#56414=CARTESIAN_POINT('Ctrl Pts',(16.2486837569799,-19.5658429540043,-7.3357800688507));
#56415=CARTESIAN_POINT('Ctrl Pts',(16.2287250388403,-19.4850344572077,-7.33991289645232));
#56416=CARTESIAN_POINT('Ctrl Pts',(16.2127296214478,-19.4033242264923,-7.34404572405394));
#56417=CARTESIAN_POINT('Ctrl Pts',(16.2007537416511,-19.3211387199432,-7.34817855165555));
#56418=CARTESIAN_POINT('Ctrl Pts',(16.1887593096482,-19.2388258972814,-7.35231778154836));
#56419=CARTESIAN_POINT('Ctrl Pts',(16.180796886798,-19.1560367972438,-7.35645701144116));
#56420=CARTESIAN_POINT('Ctrl Pts',(16.176870697397,-19.0732011954116,-7.36059624133396));
#56421=CARTESIAN_POINT('Ctrl Pts',(16.1749377014765,-19.0324184251309,-7.36263412429881));
#56422=CARTESIAN_POINT('Ctrl Pts',(16.1739822581149,-18.9916243590029,-7.36467200726366));
#56423=CARTESIAN_POINT('Ctrl Pts',(16.1740002494514,-18.9508698712832,-7.36670989022851));
#56424=CARTESIAN_POINT('Origin',(18.734,-18.952,1.76670989022851));
#56425=CARTESIAN_POINT('',(20.293535888361,-16.9218650751948,-6.05008448366249));
#56426=CARTESIAN_POINT('',(20.2954006764134,-16.9194747298048,-6.11677130171703));
#56427=CARTESIAN_POINT('',(20.293535888361,-16.9218650751948,1.76670989022851));
#56428=CARTESIAN_POINT('',(16.1740008768645,-18.954118854712,-6.6332901097715));
#56429=CARTESIAN_POINT('Ctrl Pts',(20.2954006764134,-16.9194747298048,-6.11677130171703));
#56430=CARTESIAN_POINT('Ctrl Pts',(20.8926533917614,-17.3857070907967,-6.15458085831207));
#56431=CARTESIAN_POINT('Ctrl Pts',(21.7124083657865,-18.9714392500858,-6.23478235046759));
#56432=CARTESIAN_POINT('Ctrl Pts',(20.4337935871551,-21.4567938704141,-6.35737577818358));
#56433=CARTESIAN_POINT('Ctrl Pts',(17.5479307767974,-21.7370548235123,-6.48455158486502));
#56434=CARTESIAN_POINT('Ctrl Pts',(16.247850859816,-20.0919179750469,-6.57652302872766));
#56435=CARTESIAN_POINT('Ctrl Pts',(16.1710772471096,-19.0983559299756,-6.62610253702982));
#56436=CARTESIAN_POINT('Ctrl Pts',(16.1723626618067,-18.9541202106264,-6.6332901097715));
#56437=CARTESIAN_POINT('Ctrl Pts',(16.1740008768645,-18.954118854712,-6.6332901097715));
#56438=CARTESIAN_POINT('Ctrl Pts',(16.1739325519701,-18.8715687540989,-6.63740642252224));
#56439=CARTESIAN_POINT('Ctrl Pts',(16.1778613169669,-18.7888758591841,-6.64152273527298));
#56440=CARTESIAN_POINT('Ctrl Pts',(16.1858020059738,-18.7064659224448,-6.64563904802372));
#56441=CARTESIAN_POINT('Ctrl Pts',(16.1937337220434,-18.624149108506,-6.64975070936243));
#56442=CARTESIAN_POINT('Ctrl Pts',(16.2056683130375,-18.5421150878493,-6.65386237070115));
#56443=CARTESIAN_POINT('Ctrl Pts',(16.2215685692311,-18.4607889397778,-6.65797403203986));
#56444=CARTESIAN_POINT('Ctrl Pts',(16.2374592000152,-18.3795120234588,-6.6620832043354));
#56445=CARTESIAN_POINT('Ctrl Pts',(16.2573106430753,-18.2989425946372,-6.66619237663094));
#56446=CARTESIAN_POINT('Ctrl Pts',(16.2810340922893,-18.219498630985,-6.67030154892649));
#56447=CARTESIAN_POINT('Ctrl Pts',(16.3047507902538,-18.1400772755974,-6.67440955182854));
#56448=CARTESIAN_POINT('Ctrl Pts',(16.3323371713263,-18.0617812045222,-6.67851755473059));
#56449=CARTESIAN_POINT('Ctrl Pts',(16.3636541468014,-17.9850147176797,-6.68262555763264));
#56450=CARTESIAN_POINT('Ctrl Pts',(16.3949722554067,-17.9082454532245,-6.686733709173));
#56451=CARTESIAN_POINT('Ctrl Pts',(16.4300210447237,-17.8330063217983,-6.69084186071336));
#56452=CARTESIAN_POINT('Ctrl Pts',(16.4686133150906,-17.7596815996408,-6.69495001225373));
#56453=CARTESIAN_POINT('Ctrl Pts',(16.5072438266208,-17.6862842198592,-6.69906223457025));
#56454=CARTESIAN_POINT('Ctrl Pts',(16.5494246053548,-17.6148054564872,-6.70317445688677));
#56455=CARTESIAN_POINT('Ctrl Pts',(16.5949228757402,-17.5456042319217,-6.70728667920329));
#56456=CARTESIAN_POINT('Ctrl Pts',(16.6404458510681,-17.4763654320318,-6.71140113440064));
#56457=CARTESIAN_POINT('Ctrl Pts',(16.6892896206455,-17.4094070139063,-6.71551558959799));
#56458=CARTESIAN_POINT('Ctrl Pts',(16.7411800554791,-17.3450561090319,-6.71963004479534));
#56459=CARTESIAN_POINT('Ctrl Pts',(16.7931561866084,-17.2805989295773,-6.72375129495539));
#56460=CARTESIAN_POINT('Ctrl Pts',(16.8481887081044,-17.2187582108671,-6.72787254511545));
#56461=CARTESIAN_POINT('Ctrl Pts',(16.9059658904507,-17.1598249822285,-6.73199379527551));
#56462=CARTESIAN_POINT('Ctrl Pts',(16.9382542996129,-17.1268905239829,-6.73429692959297));
#56463=CARTESIAN_POINT('Ctrl Pts',(16.9713992632832,-17.0948633881751,-6.73660006391043));
#56464=CARTESIAN_POINT('Ctrl Pts',(17.0053421035808,-17.0637887096123,-6.73890319822789));
#56465=CARTESIAN_POINT('Ctrl Pts',(17.067013876621,-17.0073281863675,-6.74308783262094));
#56466=CARTESIAN_POINT('Ctrl Pts',(17.1315694533285,-16.9537872066973,-6.74727246701399));
#56467=CARTESIAN_POINT('Ctrl Pts',(17.1987010234279,-16.9034744198481,-6.75145710140704));
#56468=CARTESIAN_POINT('Ctrl Pts',(17.2657370400465,-16.8532332470235,-6.75563577949098));
#56469=CARTESIAN_POINT('Ctrl Pts',(17.3353414020479,-16.8062114135714,-6.75981445757493));
#56470=CARTESIAN_POINT('Ctrl Pts',(17.4071710083241,-16.7626793686515,-6.76399313565888));
#56471=CARTESIAN_POINT('Ctrl Pts',(17.4802881086698,-16.7183670431123,-6.76824671354431));
#56472=CARTESIAN_POINT('Ctrl Pts',(17.5557106573434,-16.6776711711575,-6.77250029142975));
#56473=CARTESIAN_POINT('Ctrl Pts',(17.6330432222704,-16.6408327248831,-6.77675386931519));
#56474=CARTESIAN_POINT('Ctrl Pts',(17.7088765445242,-16.604708463774,-6.78092498329314));
#56475=CARTESIAN_POINT('Ctrl Pts',(17.7865460506905,-16.5722936025648,-6.78509609727109));
#56476=CARTESIAN_POINT('Ctrl Pts',(17.8656529884828,-16.5437696398415,-6.78926721124905));
#56477=CARTESIAN_POINT('Ctrl Pts',(17.9447333811781,-16.5152552486094,-6.79343692556942));
#56478=CARTESIAN_POINT('Ctrl Pts',(18.0252498151569,-16.4906293187766,-6.79760663988979));
#56479=CARTESIAN_POINT('Ctrl Pts',(18.1067845307988,-16.4700248278448,-6.80177635421016));
#56480=CARTESIAN_POINT('Ctrl Pts',(18.1883163450857,-16.4494210701093,-6.80594592015421));
#56481=CARTESIAN_POINT('Ctrl Pts',(18.2708659227711,-16.4328385786397,-6.81011548609825));
#56482=CARTESIAN_POINT('Ctrl Pts',(18.354002682145,-16.4203598126071,-6.81428505204229));
#56483=CARTESIAN_POINT('Ctrl Pts',(18.4400624274181,-16.407442308555,-6.81860121478121));
#56484=CARTESIAN_POINT('Ctrl Pts',(18.5267508916661,-16.3989225513938,-6.82291737752013));
#56485=CARTESIAN_POINT('Ctrl Pts',(18.6135836740997,-16.3948336173693,-6.82723354025905));
#56486=CARTESIAN_POINT('Ctrl Pts',(18.6975878877789,-16.3908778799405,-6.83140910445074));
#56487=CARTESIAN_POINT('Ctrl Pts',(18.7817266907703,-16.3910686822566,-6.83558466864242));
#56488=CARTESIAN_POINT('Ctrl Pts',(18.8655624783158,-16.3953828377523,-6.8397602328341));
#56489=CARTESIAN_POINT('Ctrl Pts',(18.9536326121895,-16.3999148909862,-6.84414669484664));
#56490=CARTESIAN_POINT('Ctrl Pts',(19.0413677347567,-16.4089977253144,-6.84853315685917));
#56491=CARTESIAN_POINT('Ctrl Pts',(19.1282700391328,-16.4225433120446,-6.85291961887171));
#56492=CARTESIAN_POINT('Ctrl Pts',(19.215172343509,-16.4360888987749,-6.85730608088425));
#56493=CARTESIAN_POINT('Ctrl Pts',(19.3012412773527,-16.4540970446291,-6.86169254289679));
#56494=CARTESIAN_POINT('Ctrl Pts',(19.3859971465594,-16.4764193164273,-6.86607900490932));
#56495=CARTESIAN_POINT('Ctrl Pts',(19.4675566079707,-16.4978997458344,-6.87030003977797));
#56496=CARTESIAN_POINT('Ctrl Pts',(19.5482065113869,-16.5234553484004,-6.87452107464661));
#56497=CARTESIAN_POINT('Ctrl Pts',(19.6275095404914,-16.5529917255143,-6.87874210951525));
#56498=CARTESIAN_POINT('Ctrl Pts',(19.7060066097554,-16.5822279232523,-6.88292024583855));
#56499=CARTESIAN_POINT('Ctrl Pts',(19.7831836026446,-16.6153642261603,-6.88709838216186));
#56500=CARTESIAN_POINT('Ctrl Pts',(19.8586276869387,-16.6522581523634,-6.89127651848516));
#56501=CARTESIAN_POINT('Ctrl Pts',(19.9352336917231,-16.6897202849305,-6.89551900262647));
#56502=CARTESIAN_POINT('Ctrl Pts',(20.0100524891745,-16.7310566538662,-6.89976148676778));
#56503=CARTESIAN_POINT('Ctrl Pts',(20.0826708318901,-16.7760664102025,-6.90400397090909));
#56504=CARTESIAN_POINT('Ctrl Pts',(20.1552891746057,-16.8210761665388,-6.90824645505041));
#56505=CARTESIAN_POINT('Ctrl Pts',(20.2257066150957,-16.8697590872399,-6.91248893919172));
#56506=CARTESIAN_POINT('Ctrl Pts',(20.293535888361,-16.9218650751948,-6.91673142333303));
#56507=CARTESIAN_POINT('',(16.174000571626,-18.9502892327451,-6.56670989025839));
#56508=CARTESIAN_POINT('Ctrl Pts',(16.174000571626,-18.9502892327451,-6.56670989025839));
#56509=CARTESIAN_POINT('Ctrl Pts',(16.1740643617891,-18.8548333601137,-6.57143929947809));
#56510=CARTESIAN_POINT('Ctrl Pts',(16.1794711562484,-18.7595846663132,-6.57616870869779));
#56511=CARTESIAN_POINT('Ctrl Pts',(16.1901275024526,-18.6650980721186,-6.58089811791749));
#56512=CARTESIAN_POINT('Ctrl Pts',(16.2008364140088,-18.5701453968694,-6.585650856246));
#56513=CARTESIAN_POINT('Ctrl Pts',(16.2168466650978,-18.4759625571763,-6.59040359457451));
#56514=CARTESIAN_POINT('Ctrl Pts',(16.2380139506878,-18.3830943473309,-6.59515633290303));
#56515=CARTESIAN_POINT('Ctrl Pts',(16.2593038089219,-18.2896883688619,-6.59993659274351));
#56516=CARTESIAN_POINT('Ctrl Pts',(16.2858104835345,-18.19761248234,-6.604716852584));
#56517=CARTESIAN_POINT('Ctrl Pts',(16.3173390825673,-18.1073994967126,-6.60949711242449));
#56518=CARTESIAN_POINT('Ctrl Pts',(16.3253523527945,-18.0844710744544,-6.61071205742785));
#56519=CARTESIAN_POINT('Ctrl Pts',(16.333689786842,-18.0616628735359,-6.61192700243122));
#56520=CARTESIAN_POINT('Ctrl Pts',(16.3423477078173,-18.0389833992214,-6.61314194743458));
#56521=CARTESIAN_POINT('Ctrl Pts',(16.3721681801721,-17.9608684985717,-6.61732658182763));
#56522=CARTESIAN_POINT('Ctrl Pts',(16.405875193857,-17.8840707367779,-6.62151121622068));
#56523=CARTESIAN_POINT('Ctrl Pts',(16.4433319467771,-17.8090039939072,-6.62569585061373));
#56524=CARTESIAN_POINT('Ctrl Pts',(16.4807353846456,-17.7340440992537,-6.62987452869767));
#56525=CARTESIAN_POINT('Ctrl Pts',(16.5218777565726,-17.6608107375732,-6.63405320678161));
#56526=CARTESIAN_POINT('Ctrl Pts',(16.5665735905076,-17.5896994606788,-6.63823188486555));
#56527=CARTESIAN_POINT('Ctrl Pts',(16.6120705651436,-17.5173135652528,-6.64248546275099));
#56528=CARTESIAN_POINT('Ctrl Pts',(16.661249474465,-17.4471270300731,-6.64673904063642));
#56529=CARTESIAN_POINT('Ctrl Pts',(16.7138648542455,-17.3795325145214,-6.65099261852186));
#56530=CARTESIAN_POINT('Ctrl Pts',(16.7654601822184,-17.3132484505536,-6.65516373249981));
#56531=CARTESIAN_POINT('Ctrl Pts',(16.8203596287512,-17.2494571801029,-6.65933484647776));
#56532=CARTESIAN_POINT('Ctrl Pts',(16.8782881026493,-17.1884996869773,-6.66350596045572));
#56533=CARTESIAN_POINT('Ctrl Pts',(16.9361971380885,-17.1275626487273,-6.66767567477609));
#56534=CARTESIAN_POINT('Ctrl Pts',(16.99713286563,-17.0694578324917,-6.67184538909646));
#56535=CARTESIAN_POINT('Ctrl Pts',(17.060781453689,-17.0144913687209,-6.67601510341684));
#56536=CARTESIAN_POINT('Ctrl Pts',(17.1244277768581,-16.9595268608928,-6.68018466936088));
#56537=CARTESIAN_POINT('Ctrl Pts',(17.1907864198799,-16.9077007835217,-6.68435423530492));
#56538=CARTESIAN_POINT('Ctrl Pts',(17.2595094445542,-16.8592798558094,-6.68852380124897));
#56539=CARTESIAN_POINT('Ctrl Pts',(17.3306486859969,-16.8091565080125,-6.69283996398789));
#56540=CARTESIAN_POINT('Ctrl Pts',(17.4043212347439,-16.7626825189769,-6.69715612672681));
#56541=CARTESIAN_POINT('Ctrl Pts',(17.4801089073792,-16.7201045885064,-6.70147228946573));
#56542=CARTESIAN_POINT('Ctrl Pts',(17.55342780455,-16.6789136296426,-6.70564785365741));
#56543=CARTESIAN_POINT('Ctrl Pts',(17.6287256988456,-16.6413689670528,-6.70982341784909));
#56544=CARTESIAN_POINT('Ctrl Pts',(17.7056010183993,-16.6076460304291,-6.71399898204077));
#56545=CARTESIAN_POINT('Ctrl Pts',(17.78635912759,-16.5722198284453,-6.71838544405331));
#56546=CARTESIAN_POINT('Ctrl Pts',(17.8688576552586,-16.5410117758974,-6.72277190606585));
#56547=CARTESIAN_POINT('Ctrl Pts',(17.9526121488767,-16.5141663251737,-6.7271583680784));
#56548=CARTESIAN_POINT('Ctrl Pts',(18.0363666424947,-16.48732087445,-6.73154483009094));
#56549=CARTESIAN_POINT('Ctrl Pts',(18.1213765216826,-16.4648381003647,-6.73593129210348));
#56550=CARTESIAN_POINT('Ctrl Pts',(18.20714644876,-16.4468003401833,-6.74031775411602));
#56551=CARTESIAN_POINT('Ctrl Pts',(18.2889778682176,-16.4295908639743,-6.7445027922187));
#56552=CARTESIAN_POINT('Ctrl Pts',(18.3718056859211,-16.4163630651953,-6.74868783032138));
#56553=CARTESIAN_POINT('Ctrl Pts',(18.4552077229431,-16.4072259695106,-6.75287286842406));
#56554=CARTESIAN_POINT('Ctrl Pts',(18.5384664989632,-16.3981045687601,-6.75705071782041));
#56555=CARTESIAN_POINT('Ctrl Pts',(18.6222970795582,-16.3930599483572,-6.76122856721675));
#56556=CARTESIAN_POINT('Ctrl Pts',(18.7062667332562,-16.3921502259086,-6.7654064166131));
#56557=CARTESIAN_POINT('Ctrl Pts',(18.7901543122248,-16.391241392653,-6.76958018244063));
#56558=CARTESIAN_POINT('Ctrl Pts',(18.8741802371499,-16.3944594382537,-6.77375394826816));
#56559=CARTESIAN_POINT('Ctrl Pts',(18.9579070743402,-16.4018106693697,-6.7779277140957));
#56560=CARTESIAN_POINT('Ctrl Pts',(19.041577192961,-16.4091569205853,-6.78209865251406));
#56561=CARTESIAN_POINT('Ctrl Pts',(19.124948169362,-16.4206307562896,-6.78626959093242));
#56562=CARTESIAN_POINT('Ctrl Pts',(19.2075843584854,-16.4361864426397,-6.79044052935078));
#56563=CARTESIAN_POINT('Ctrl Pts',(19.2901893576105,-16.4517362576901,-6.79460989350049));
#56564=CARTESIAN_POINT('Ctrl Pts',(19.3720596691157,-16.471364776407,-6.7987792576502));
#56565=CARTESIAN_POINT('Ctrl Pts',(19.4527679051966,-16.4949748274673,-6.80294862179992));
#56566=CARTESIAN_POINT('Ctrl Pts',(19.5335042821171,-16.5185931107316,-6.80711943969727));
#56567=CARTESIAN_POINT('Ctrl Pts',(19.6130773298815,-16.5461955784803,-6.81129025759462));
#56568=CARTESIAN_POINT('Ctrl Pts',(19.6910737323175,-16.5776348488685,-6.81546107549197));
#56569=CARTESIAN_POINT('Ctrl Pts',(19.7690820104975,-16.6090789062047,-6.81963252843869));
#56570=CARTESIAN_POINT('Ctrl Pts',(19.8455127429621,-16.64436074602,-6.8238039813854));
#56571=CARTESIAN_POINT('Ctrl Pts',(19.9199734317183,-16.6832851613175,-6.82797543433211));
#56572=CARTESIAN_POINT('Ctrl Pts',(19.9945177108395,-16.7222532735795,-6.83215157019648));
#56573=CARTESIAN_POINT('Ctrl Pts',(20.0670871265703,-16.7648719041894,-6.83632770606085));
#56574=CARTESIAN_POINT('Ctrl Pts',(20.1373150369702,-16.8109005378046,-6.84050384192522));
#56575=CARTESIAN_POINT('Ctrl Pts',(20.1907958241465,-16.8459528061175,-6.84368410219653));
#56576=CARTESIAN_POINT('Ctrl Pts',(20.2429192181243,-16.8829816922142,-6.84686436246784));
#56577=CARTESIAN_POINT('Ctrl Pts',(20.293535888361,-16.9218650751948,-6.85004462273914));
#56578=CARTESIAN_POINT('Ctrl Pts',(20.293535888361,-16.9218650751948,-6.05008448366249));
#56579=CARTESIAN_POINT('Ctrl Pts',(20.3602243278818,-16.9730946824,-6.05425482454861));
#56580=CARTESIAN_POINT('Ctrl Pts',(20.4243678404919,-17.0275998935312,-6.05842516543473));
#56581=CARTESIAN_POINT('Ctrl Pts',(20.4856397847705,-17.0850886297391,-6.06259550632085));
#56582=CARTESIAN_POINT('Ctrl Pts',(20.5469803613649,-17.1426417605921,-6.06677051851546));
#56583=CARTESIAN_POINT('Ctrl Pts',(20.6054426153629,-17.20318476991,-6.07094553071006));
#56584=CARTESIAN_POINT('Ctrl Pts',(20.6607367305677,-17.2663886654744,-6.07512054290466));
#56585=CARTESIAN_POINT('Ctrl Pts',(20.7160670517863,-17.3296339462947,-6.07929828885399));
#56586=CARTESIAN_POINT('Ctrl Pts',(20.7682248206514,-17.3955432204527,-6.08347603480332));
#56587=CARTESIAN_POINT('Ctrl Pts',(20.8169619670476,-17.4637562552346,-6.08765378075265));
#56588=CARTESIAN_POINT('Ctrl Pts',(20.8657776958325,-17.5320792747738,-6.09183826278073));
#56589=CARTESIAN_POINT('Ctrl Pts',(20.9111615486972,-17.6027130808414,-6.09602274480881));
#56590=CARTESIAN_POINT('Ctrl Pts',(20.9529102925223,-17.6752709317405,-6.10020722683688));
#56591=CARTESIAN_POINT('Ctrl Pts',(20.9669828868101,-17.6997286065002,-6.1016177247942));
#56592=CARTESIAN_POINT('Ctrl Pts',(20.980642853236,-17.7244047147345,-6.10302822275152));
#56593=CARTESIAN_POINT('Ctrl Pts',(20.9938836431733,-17.7492839406918,-6.10443872070884));
#56594=CARTESIAN_POINT('Ctrl Pts',(21.0331661282527,-17.8230950824048,-6.10862335510189));
#56595=CARTESIAN_POINT('Ctrl Pts',(21.0689017421373,-17.8989701434485,-6.11280798949494));
#56596=CARTESIAN_POINT('Ctrl Pts',(21.1008684225543,-17.9765340240093,-6.11699262388799));
#56597=CARTESIAN_POINT('Ctrl Pts',(21.1327896023584,-18.0539875019867,-6.12117130197194));
#56598=CARTESIAN_POINT('Ctrl Pts',(21.1609523307068,-18.1331246030379,-6.12534998005589));
#56599=CARTESIAN_POINT('Ctrl Pts',(21.1851803441784,-18.2135455868415,-6.12952865813984));
#56600=CARTESIAN_POINT('Ctrl Pts',(21.2098426273792,-18.2954080589821,-6.13378223602527));
#56601=CARTESIAN_POINT('Ctrl Pts',(21.2304275222058,-18.3786004681764,-6.13803581391071));
#56602=CARTESIAN_POINT('Ctrl Pts',(21.2468003698023,-18.4626797556596,-6.14228939179614));
#56603=CARTESIAN_POINT('Ctrl Pts',(21.2628557977992,-18.5451290020877,-6.14646050577409));
#56604=CARTESIAN_POINT('Ctrl Pts',(21.2748609466779,-18.6284305735959,-6.15063161975205));
#56605=CARTESIAN_POINT('Ctrl Pts',(21.2827395777799,-18.7121530390891,-6.15480273373));
#56606=CARTESIAN_POINT('Ctrl Pts',(21.2906155651312,-18.7958474107005,-6.15897244805037));
#56607=CARTESIAN_POINT('Ctrl Pts',(21.2943677416632,-18.8799619381738,-6.16314216237074));
#56608=CARTESIAN_POINT('Ctrl Pts',(21.2939715980996,-18.9640588939549,-6.16731187669111));
#56609=CARTESIAN_POINT('Ctrl Pts',(21.2935754686324,-19.0481528572055,-6.17148144263516));
#56610=CARTESIAN_POINT('Ctrl Pts',(21.2890313155854,-19.1322287899834,-6.1756510085792));
#56611=CARTESIAN_POINT('Ctrl Pts',(21.2803667494581,-19.2158491562509,-6.17982057452325));
#56612=CARTESIAN_POINT('Ctrl Pts',(21.2713975478746,-19.3024095114395,-6.18413673726217));
#56613=CARTESIAN_POINT('Ctrl Pts',(21.2580128490967,-19.388481144016,-6.18845290000109));
#56614=CARTESIAN_POINT('Ctrl Pts',(21.2403015155518,-19.4735867263868,-6.19276906274001));
#56615=CARTESIAN_POINT('Ctrl Pts',(21.2231671268342,-19.5559200033636,-6.19694462693169));
#56616=CARTESIAN_POINT('Ctrl Pts',(21.2019838191122,-19.6373487577952,-6.20112019112337));
#56617=CARTESIAN_POINT('Ctrl Pts',(21.1768832583851,-19.7174550188626,-6.20529575531505));
#56618=CARTESIAN_POINT('Ctrl Pts',(21.1505149280065,-19.801607256742,-6.20968221732759));
#56619=CARTESIAN_POINT('Ctrl Pts',(21.1198234271564,-19.8842993445549,-6.21406867934013));
#56620=CARTESIAN_POINT('Ctrl Pts',(21.0850182368018,-19.965071197017,-6.21845514135266));
#56621=CARTESIAN_POINT('Ctrl Pts',(21.0502130464472,-20.045843049479,-6.2228416033652));
#56622=CARTESIAN_POINT('Ctrl Pts',(21.0112944915984,-20.1246941799628,-6.22722806537774));
#56623=CARTESIAN_POINT('Ctrl Pts',(20.9685260259017,-20.2011971179794,-6.23161452739027));
#56624=CARTESIAN_POINT('Ctrl Pts',(20.9277254007097,-20.2741800424132,-6.23579916178332));
#56625=CARTESIAN_POINT('Ctrl Pts',(20.883269491877,-20.3452977698653,-6.23998379617637));
#56626=CARTESIAN_POINT('Ctrl Pts',(20.8353535008893,-20.4141605466913,-6.24416843056941));
#56627=CARTESIAN_POINT('Ctrl Pts',(20.7875057123839,-20.482925305878,-6.24834710865336));
#56628=CARTESIAN_POINT('Ctrl Pts',(20.7362078848242,-20.5494411154157,-6.25252578673731));
#56629=CARTESIAN_POINT('Ctrl Pts',(20.6817007285136,-20.6133433938074,-6.25670446482125));
#56630=CARTESIAN_POINT('Ctrl Pts',(20.6262165705998,-20.6783910746135,-6.26095804270669));
#56631=CARTESIAN_POINT('Ctrl Pts',(20.5674071330978,-20.7407301867605,-6.26521162059212));
#56632=CARTESIAN_POINT('Ctrl Pts',(20.5055720700286,-20.8000076841547,-6.26946519847756));
#56633=CARTESIAN_POINT('Ctrl Pts',(20.4449358003181,-20.8581359715914,-6.27363631245551));
#56634=CARTESIAN_POINT('Ctrl Pts',(20.3813905208317,-20.9133199626604,-6.27780742643346));
#56635=CARTESIAN_POINT('Ctrl Pts',(20.3152577303048,-20.9652620272462,-6.28197854041141));
#56636=CARTESIAN_POINT('Ctrl Pts',(20.2491471312743,-21.0171866621706,-6.28614825473179));
#56637=CARTESIAN_POINT('Ctrl Pts',(20.1804511070729,-21.0658712472024,-6.29031796905216));
#56638=CARTESIAN_POINT('Ctrl Pts',(20.1095244508952,-21.1110582402958,-6.29448768337254));
#56639=CARTESIAN_POINT('Ctrl Pts',(20.0386003185924,-21.1562436254421,-6.29865724931658));
#56640=CARTESIAN_POINT('Ctrl Pts',(19.9654461005735,-21.1979314196438,-6.30282681526062));
#56641=CARTESIAN_POINT('Ctrl Pts',(19.8904446404442,-21.235908009003,-6.30699638120466));
#56642=CARTESIAN_POINT('Ctrl Pts',(19.812806221501,-21.2752198083949,-6.31131254394358));
#56643=CARTESIAN_POINT('Ctrl Pts',(19.7331887160477,-21.3105543371331,-6.3156287066825));
#56644=CARTESIAN_POINT('Ctrl Pts',(19.6520415805983,-21.3417279460835,-6.31994486942142));
#56645=CARTESIAN_POINT('Ctrl Pts',(19.573537804551,-21.3718860780012,-6.32412043361311));
#56646=CARTESIAN_POINT('Ctrl Pts',(19.493602985757,-21.3981501088936,-6.32829599780479));
#56647=CARTESIAN_POINT('Ctrl Pts',(19.4126598398381,-21.4204045093523,-6.33247156199647));
#56648=CARTESIAN_POINT('Ctrl Pts',(19.3276284480429,-21.4437829266734,-6.33685802400901));
#56649=CARTESIAN_POINT('Ctrl Pts',(19.2414847611989,-21.4627358902474,-6.34124448602155));
#56650=CARTESIAN_POINT('Ctrl Pts',(19.1547290262948,-21.4771905049784,-6.3456309480341));
#56651=CARTESIAN_POINT('Ctrl Pts',(19.0679732913907,-21.4916451197093,-6.35001741004664));
#56652=CARTESIAN_POINT('Ctrl Pts',(18.9806060935248,-21.5016013954773,-6.35440387205918));
#56653=CARTESIAN_POINT('Ctrl Pts',(18.8931294701917,-21.5070494734381,-6.35879033407172));
#56654=CARTESIAN_POINT('Ctrl Pts',(18.8096777759696,-21.512246877256,-6.36297496846477));
#56655=CARTESIAN_POINT('Ctrl Pts',(18.7258158815286,-21.5133611702432,-6.36715960285781));
#56656=CARTESIAN_POINT('Ctrl Pts',(18.6419771668657,-21.5103455197025,-6.37134423725086));
#56657=CARTESIAN_POINT('Ctrl Pts',(18.5582577862359,-21.5073341615672,-6.3755229153348));
#56658=CARTESIAN_POINT('Ctrl Pts',(18.4745619756521,-21.5002045527773,-6.37970159341874));
#56659=CARTESIAN_POINT('Ctrl Pts',(18.3913265823787,-21.4889617515555,-6.38388027150268));
#56660=CARTESIAN_POINT('Ctrl Pts',(18.306599254501,-21.4775174312019,-6.38813384938812));
#56661=CARTESIAN_POINT('Ctrl Pts',(18.2223494934531,-21.4618109801083,-6.39238742727355));
#56662=CARTESIAN_POINT('Ctrl Pts',(18.1390363521672,-21.4419032627308,-6.39664100515899));
#56663=CARTESIAN_POINT('Ctrl Pts',(18.0573383986974,-21.4223814953014,-6.40081211913694));
#56664=CARTESIAN_POINT('Ctrl Pts',(17.9765415407097,-21.3988200192303,-6.4049832331149));
#56665=CARTESIAN_POINT('Ctrl Pts',(17.8970700591984,-21.3713280625392,-6.40915434709285));
#56666=CARTESIAN_POINT('Ctrl Pts',(17.8176252451101,-21.3438453310398,-6.41332406141322));
#56667=CARTESIAN_POINT('Ctrl Pts',(17.739505358624,-21.3124348885694,-6.41749377573359));
#56668=CARTESIAN_POINT('Ctrl Pts',(17.6631189946706,-21.2772556574331,-6.42166349005396));
#56669=CARTESIAN_POINT('Ctrl Pts',(17.5867353488719,-21.2420776781248,-6.425833055998));
#56670=CARTESIAN_POINT('Ctrl Pts',(17.5120855204506,-21.2031313700067,-6.43000262194204));
#56671=CARTESIAN_POINT('Ctrl Pts',(17.4395563508724,-21.1606230188136,-6.43417218788608));
#56672=CARTESIAN_POINT('Ctrl Pts',(17.364477145166,-21.1166201264321,-6.438488350625));
#56673=CARTESIAN_POINT('Ctrl Pts',(17.291670952671,-21.068800314323,-6.44280451336393));
#56674=CARTESIAN_POINT('Ctrl Pts',(17.2215354755327,-21.0174420984932,-6.44712067610285));
#56675=CARTESIAN_POINT('Ctrl Pts',(17.1536846541853,-20.9677568711422,-6.45129624029452));
#56676=CARTESIAN_POINT('Ctrl Pts',(17.0883335592485,-20.9147605602812,-6.4554718044862));
#56677=CARTESIAN_POINT('Ctrl Pts',(17.0258081406203,-20.8587460689743,-6.45964736867787));
#56678=CARTESIAN_POINT('Ctrl Pts',(16.9601247117371,-20.7999024188732,-6.46403383069042));
#56679=CARTESIAN_POINT('Ctrl Pts',(16.8975603248984,-20.7377280904825,-6.46842029270297));
#56680=CARTESIAN_POINT('Ctrl Pts',(16.838447047551,-20.6726042556212,-6.47280675471551));
#56681=CARTESIAN_POINT('Ctrl Pts',(16.7793337702036,-20.6074804207598,-6.47719321672806));
#56682=CARTESIAN_POINT('Ctrl Pts',(16.7236719107426,-20.5394075767508,-6.48157967874061));
#56683=CARTESIAN_POINT('Ctrl Pts',(16.6717415022696,-20.4688025212726,-6.48596614075316));
#56684=CARTESIAN_POINT('Ctrl Pts',(16.6219091295864,-20.4010499743281,-6.49017538570612));
#56685=CARTESIAN_POINT('Ctrl Pts',(16.5753265021952,-20.3307132360493,-6.49438463065908));
#56686=CARTESIAN_POINT('Ctrl Pts',(16.532270626113,-20.2581346654013,-6.49859387561204));
#56687=CARTESIAN_POINT('Ctrl Pts',(16.489277141859,-20.1856612676153,-6.50279702099133));
#56688=CARTESIAN_POINT('Ctrl Pts',(16.4498004872776,-20.110952875341,-6.50700016637061));
#56689=CARTESIAN_POINT('Ctrl Pts',(16.4140760664827,-20.0343829926109,-6.5112033117499));
#56690=CARTESIAN_POINT('Ctrl Pts',(16.3783931208862,-19.9579020056842,-6.51540157737789));
#56691=CARTESIAN_POINT('Ctrl Pts',(16.3464539443372,-19.8795642299173,-6.51959984300589));
#56692=CARTESIAN_POINT('Ctrl Pts',(16.3184487740251,-19.7997689984254,-6.52379810863388));
#56693=CARTESIAN_POINT('Ctrl Pts',(16.2904693914727,-19.7200472440891,-6.52799250840909));
#56694=CARTESIAN_POINT('Ctrl Pts',(16.2664169618497,-19.6388711282231,-6.5321869081843));
#56695=CARTESIAN_POINT('Ctrl Pts',(16.2464336691667,-19.5566600282013,-6.53638130795952));
#56696=CARTESIAN_POINT('Ctrl Pts',(16.2264610773219,-19.4744929513394,-6.54057346167876));
#56697=CARTESIAN_POINT('Ctrl Pts',(16.210553397436,-19.3912924312907,-6.54476561539801));
#56698=CARTESIAN_POINT('Ctrl Pts',(16.1988026788696,-19.3074919730929,-6.54895776911726));
#56699=CARTESIAN_POINT('Ctrl Pts',(16.1870533030452,-19.2237010906829,-6.55314944380363));
#56700=CARTESIAN_POINT('Ctrl Pts',(16.1794600117858,-19.1393108539568,-6.55734111849));
#56701=CARTESIAN_POINT('Ctrl Pts',(16.1760633700115,-19.0547628189716,-6.56153279317637));
#56702=CARTESIAN_POINT('Ctrl Pts',(16.1746649834927,-19.0199546642812,-6.56325849219375));
#56703=CARTESIAN_POINT('Ctrl Pts',(16.173977295445,-18.9851198216844,-6.56498419121113));
#56704=CARTESIAN_POINT('Ctrl Pts',(16.1740005716256,-18.9502892333483,-6.5667098902285));
#56705=CARTESIAN_POINT('Origin',(18.734,-18.952,1.76670989022851));
#56706=CARTESIAN_POINT('',(20.293535888361,-16.9218650751948,-5.25018234329749));
#56707=CARTESIAN_POINT('',(20.293535888361,-16.9218650751948,-5.31661775147474));
#56708=CARTESIAN_POINT('',(20.293535888361,-16.9218650751948,1.76670989022851));
#56709=CARTESIAN_POINT('',(16.1740005630998,-18.9503020392334,-5.8332901097715));
#56710=CARTESIAN_POINT('Ctrl Pts',(20.293535888361,-16.9218650751948,-5.31661775147473));
#56711=CARTESIAN_POINT('Ctrl Pts',(20.3601996645773,-16.9730757362167,-5.32080132225747));
#56712=CARTESIAN_POINT('Ctrl Pts',(20.424260063449,-17.0275132017657,-5.32498489304021));
#56713=CARTESIAN_POINT('Ctrl Pts',(20.4854058706178,-17.0848691860597,-5.32916846382294));
#56714=CARTESIAN_POINT('Ctrl Pts',(20.5380265777208,-17.1342284567911,-5.33276875079266));
#56715=CARTESIAN_POINT('Ctrl Pts',(20.5884892430759,-17.185748417461,-5.33636903776239));
#56716=CARTESIAN_POINT('Ctrl Pts',(20.6366195645771,-17.239213150305,-5.33996932473211));
#56717=CARTESIAN_POINT('Ctrl Pts',(20.6925617159657,-17.3013555188871,-5.34415395912515));
#56718=CARTESIAN_POINT('Ctrl Pts',(20.7455602793472,-17.3663571440021,-5.3483385935182));
#56719=CARTESIAN_POINT('Ctrl Pts',(20.7953091936645,-17.4339076417706,-5.35252322791125));
#56720=CARTESIAN_POINT('Ctrl Pts',(20.8449872965599,-17.5013619897667,-5.35670190599519));
#56721=CARTESIAN_POINT('Ctrl Pts',(20.8914246675681,-17.5713576368076,-5.36088058407914));
#56722=CARTESIAN_POINT('Ctrl Pts',(20.934353739878,-17.6435492292773,-5.36505926216309));
#56723=CARTESIAN_POINT('Ctrl Pts',(20.9780522849565,-17.7170348041588,-5.36931284004852));
#56724=CARTESIAN_POINT('Ctrl Pts',(21.0181151991573,-17.7927954651137,-5.37356641793396));
#56725=CARTESIAN_POINT('Ctrl Pts',(21.0543048298795,-17.8704337762126,-5.37781999581939));
#56726=CARTESIAN_POINT('Ctrl Pts',(21.089792853992,-17.9465669171521,-5.38199110979734));
#56727=CARTESIAN_POINT('Ctrl Pts',(21.1215562334332,-18.0245051179384,-5.38616222377529));
#56728=CARTESIAN_POINT('Ctrl Pts',(21.1494168148284,-18.1038481205325,-5.39033333775325));
#56729=CARTESIAN_POINT('Ctrl Pts',(21.1772680473364,-18.1831644988157,-5.39450305207362));
#56730=CARTESIAN_POINT('Ctrl Pts',(21.2012189304412,-18.2638843090192,-5.39867276639399));
#56731=CARTESIAN_POINT('Ctrl Pts',(21.2211399893044,-18.3455886927152,-5.40284248071437));
#56732=CARTESIAN_POINT('Ctrl Pts',(21.2410603392909,-18.4272901690186,-5.40701204665841));
#56733=CARTESIAN_POINT('Ctrl Pts',(21.2569510420043,-18.5099757020134,-5.41118161260245));
#56734=CARTESIAN_POINT('Ctrl Pts',(21.2687332465284,-18.5932140346339,-5.4153511785465));
#56735=CARTESIAN_POINT('Ctrl Pts',(21.2809296988287,-18.6793789243438,-5.41966734128542));
#56736=CARTESIAN_POINT('Ctrl Pts',(21.2887232939913,-18.7661356875971,-5.42398350402433));
#56737=CARTESIAN_POINT('Ctrl Pts',(21.2920850129342,-18.8529996636308,-5.42829966676325));
#56738=CARTESIAN_POINT('Ctrl Pts',(21.2953372242362,-18.9370340547817,-5.43247523095493));
#56739=CARTESIAN_POINT('Ctrl Pts',(21.2944419142066,-19.0211683105535,-5.43665079514661));
#56740=CARTESIAN_POINT('Ctrl Pts',(21.2894259327675,-19.1049650356758,-5.44082635933829));
#56741=CARTESIAN_POINT('Ctrl Pts',(21.2841566060302,-19.1929941341762,-5.44521282135083));
#56742=CARTESIAN_POINT('Ctrl Pts',(21.2743394628619,-19.2806501283313,-5.44959928336338));
#56743=CARTESIAN_POINT('Ctrl Pts',(21.2600666971253,-19.3674359657934,-5.45398574537592));
#56744=CARTESIAN_POINT('Ctrl Pts',(21.2457939313886,-19.4542218032555,-5.45837220738846));
#56745=CARTESIAN_POINT('Ctrl Pts',(21.2270657409798,-19.5401369333207,-5.462758669401));
#56746=CARTESIAN_POINT('Ctrl Pts',(21.2040345704695,-19.6247029215675,-5.46714513141354));
#56747=CARTESIAN_POINT('Ctrl Pts',(21.1820630982548,-19.7053779033381,-5.47132976580658));
#56748=CARTESIAN_POINT('Ctrl Pts',(21.1560941354244,-19.7851254547589,-5.47551440019963));
#56749=CARTESIAN_POINT('Ctrl Pts',(21.1262230006563,-19.8635202220089,-5.47969903459268));
#56750=CARTESIAN_POINT('Ctrl Pts',(21.0963943837511,-19.9418034040111,-5.48387771267662));
#56751=CARTESIAN_POINT('Ctrl Pts',(21.0626747898134,-20.0187372003264,-5.48805639076056));
#56752=CARTESIAN_POINT('Ctrl Pts',(21.0252097777407,-20.0939096962481,-5.49223506884451));
#56753=CARTESIAN_POINT('Ctrl Pts',(20.9870732322522,-20.1704296051336,-5.49648864672994));
#56754=CARTESIAN_POINT('Ctrl Pts',(20.9450558013773,-20.2451239847431,-5.50074222461538));
#56755=CARTESIAN_POINT('Ctrl Pts',(20.8993630289916,-20.3175778823181,-5.50499580250082));
#56756=CARTESIAN_POINT('Ctrl Pts',(20.8545561001607,-20.3886271197065,-5.50916691647877));
#56757=CARTESIAN_POINT('Ctrl Pts',(20.8062153221385,-20.4575215650235,-5.51333803045672));
#56758=CARTESIAN_POINT('Ctrl Pts',(20.7545808175508,-20.5238947673893,-5.51750914443467));
#56759=CARTESIAN_POINT('Ctrl Pts',(20.7029636394197,-20.5902456975861,-5.52167885875505));
#56760=CARTESIAN_POINT('Ctrl Pts',(20.6480552119857,-20.6540767022586,-5.52584857307542));
#56761=CARTESIAN_POINT('Ctrl Pts',(20.5901376466264,-20.7150521934351,-5.53001828739579));
#56762=CARTESIAN_POINT('Ctrl Pts',(20.5322221422225,-20.776025514842,-5.53418785333984));
#56763=CARTESIAN_POINT('Ctrl Pts',(20.4712980302309,-20.8341431918207,-5.53835741928388));
#56764=CARTESIAN_POINT('Ctrl Pts',(20.4076852490905,-20.8891054919588,-5.54252698522792));
#56765=CARTESIAN_POINT('Ctrl Pts',(20.34183592104,-20.9460001987665,-5.54684314796684));
#56766=CARTESIAN_POINT('Ctrl Pts',(20.2731057379437,-20.999513169412,-5.55115931070577));
#56767=CARTESIAN_POINT('Ctrl Pts',(20.2018865153254,-21.0493576657609,-5.55547547344469));
#56768=CARTESIAN_POINT('Ctrl Pts',(20.1329872513929,-21.0975784828839,-5.55965103763637));
#56769=CARTESIAN_POINT('Ctrl Pts',(20.0617590424853,-21.1423659457519,-5.56382660182805));
#56770=CARTESIAN_POINT('Ctrl Pts',(19.9885842021594,-21.1835058771359,-5.56800216601973));
#56771=CARTESIAN_POINT('Ctrl Pts',(19.9117134746052,-21.2267236886533,-5.57238862803227));
#56772=CARTESIAN_POINT('Ctrl Pts',(19.8326948219823,-21.2659155519541,-5.57677509004481));
#56773=CARTESIAN_POINT('Ctrl Pts',(19.7519960894443,-21.3008899424784,-5.58116155205735));
#56774=CARTESIAN_POINT('Ctrl Pts',(19.6712973569064,-21.3358643330026,-5.5855480140699));
#56775=CARTESIAN_POINT('Ctrl Pts',(19.5889191146256,-21.3666211190642,-5.58993447608244));
#56776=CARTESIAN_POINT('Ctrl Pts',(19.5053461655913,-21.393029514944,-5.59432093809498));
#56777=CARTESIAN_POINT('Ctrl Pts',(19.4256185318269,-21.4182228213827,-5.59850557248803));
#56778=CARTESIAN_POINT('Ctrl Pts',(19.3445069543659,-21.4395528703719,-5.60269020688107));
#56779=CARTESIAN_POINT('Ctrl Pts',(19.2624206826504,-21.4568695738795,-5.60687484127412));
#56780=CARTESIAN_POINT('Ctrl Pts',(19.1804512505824,-21.4741616292031,-5.61105351935807));
#56781=CARTESIAN_POINT('Ctrl Pts',(19.0975103262627,-21.4874515917235,-5.61523219744201));
#56782=CARTESIAN_POINT('Ctrl Pts',(19.0140230530432,-21.4966388918203,-5.61941087552595));
#56783=CARTESIAN_POINT('Ctrl Pts',(18.9290393304525,-21.5059908676685,-5.62366445341139));
#56784=CARTESIAN_POINT('Ctrl Pts',(18.8434899394337,-21.511091508697,-5.62791803129682));
#56785=CARTESIAN_POINT('Ctrl Pts',(18.7578350465906,-21.5118890387191,-5.63217160918226));
#56786=CARTESIAN_POINT('Ctrl Pts',(18.673840740987,-21.5126711070654,-5.63634272316021));
#56787=CARTESIAN_POINT('Ctrl Pts',(18.5897454689698,-21.5093154194064,-5.64051383713816));
#56788=CARTESIAN_POINT('Ctrl Pts',(18.5059873315596,-21.5018255279589,-5.64468495111611));
#56789=CARTESIAN_POINT('Ctrl Pts',(18.4222573000014,-21.4943381498168,-5.64885466543648));
#56790=CARTESIAN_POINT('Ctrl Pts',(18.3388646361979,-21.4827193639703,-5.65302437975686));
#56791=CARTESIAN_POINT('Ctrl Pts',(18.2562442180637,-21.4670247340387,-5.65719409407723));
#56792=CARTESIAN_POINT('Ctrl Pts',(18.1736267399184,-21.4513306625893,-5.66136366002127));
#56793=CARTESIAN_POINT('Ctrl Pts',(18.0917819045973,-21.4315611221138,-5.66553322596531));
#56794=CARTESIAN_POINT('Ctrl Pts',(18.0111349162342,-21.4078228907379,-5.66970279190935));
#56795=CARTESIAN_POINT('Ctrl Pts',(17.9276524792491,-21.3832500524311,-5.67401895464827));
#56796=CARTESIAN_POINT('Ctrl Pts',(17.8454541950085,-21.354424401291,-5.6783351173872));
#56797=CARTESIAN_POINT('Ctrl Pts',(17.7649932472177,-21.3215201862534,-5.68265128012612));
#56798=CARTESIAN_POINT('Ctrl Pts',(17.6871533063382,-21.2896878225597,-5.6868268443178));
#56799=CARTESIAN_POINT('Ctrl Pts',(17.6109396593041,-21.2540387751658,-5.69100240850948));
#56800=CARTESIAN_POINT('Ctrl Pts',(17.5367393343476,-21.2147785791989,-5.69517797270115));
#56801=CARTESIAN_POINT('Ctrl Pts',(17.458791327372,-21.173535444066,-5.6995644347137));
#56802=CARTESIAN_POINT('Ctrl Pts',(17.3830658746254,-21.1283070744553,-5.70395089672624));
#56803=CARTESIAN_POINT('Ctrl Pts',(17.3099772536615,-21.0793831854912,-5.70833735873878));
#56804=CARTESIAN_POINT('Ctrl Pts',(17.2368886326976,-21.0304592965271,-5.71272382075132));
#56805=CARTESIAN_POINT('Ctrl Pts',(17.1664372628671,-20.977840296355,-5.71711028276386));
#56806=CARTESIAN_POINT('Ctrl Pts',(17.0989955289256,-20.9218630357379,-5.72149674477641));
#56807=CARTESIAN_POINT('Ctrl Pts',(17.0355419517776,-20.8691959820086,-5.72562381401755));
#56808=CARTESIAN_POINT('Ctrl Pts',(16.9745020021859,-20.8133485129554,-5.72975088325869));
#56809=CARTESIAN_POINT('Ctrl Pts',(16.9162185170907,-20.7545732940416,-5.73387795249984));
#56810=CARTESIAN_POINT('Ctrl Pts',(16.8577217299027,-20.6955829734197,-5.73802012571949));
#56811=CARTESIAN_POINT('Ctrl Pts',(16.8020020379165,-20.6336436795684,-5.74216229893914));
#56812=CARTESIAN_POINT('Ctrl Pts',(16.7493744028763,-20.5690532580101,-5.7463044721588));
#56813=CARTESIAN_POINT('Ctrl Pts',(16.6970742796337,-20.5048647949489,-5.75042086784547));
#56814=CARTESIAN_POINT('Ctrl Pts',(16.6478281605157,-20.4380584608901,-5.75453726353214));
#56815=CARTESIAN_POINT('Ctrl Pts',(16.6019085746493,-20.3689637094668,-5.75865365921882));
#56816=CARTESIAN_POINT('Ctrl Pts',(16.5560170315913,-20.2999111537828,-5.76276754104799));
#56817=CARTESIAN_POINT('Ctrl Pts',(16.5134482524877,-20.2285733472958,-5.76688142287716));
#56818=CARTESIAN_POINT('Ctrl Pts',(16.4744330306069,-20.1553108953332,-5.77099530470634));
#56819=CARTESIAN_POINT('Ctrl Pts',(16.4354291736147,-20.0820697842618,-5.77510798818763));
#56820=CARTESIAN_POINT('Ctrl Pts',(16.3999770407453,-20.0069055590536,-5.77922067166892));
#56821=CARTESIAN_POINT('Ctrl Pts',(16.3682620211175,-19.9302043831803,-5.78333335515021));
#56822=CARTESIAN_POINT('Ctrl Pts',(16.3361584999705,-19.852563635971,-5.78749641803532));
#56823=CARTESIAN_POINT('Ctrl Pts',(16.3078844956127,-19.7733484709671,-5.79165948092042));
#56824=CARTESIAN_POINT('Ctrl Pts',(16.2835818660734,-19.6929797358388,-5.79582254380553));
#56825=CARTESIAN_POINT('Ctrl Pts',(16.2595524301165,-19.6135144512041,-5.79993880837768));
#56826=CARTESIAN_POINT('Ctrl Pts',(16.2394055983612,-19.5329218806178,-5.80405507294983));
#56827=CARTESIAN_POINT('Ctrl Pts',(16.2232275631065,-19.4516216269696,-5.80817133752197));
#56828=CARTESIAN_POINT('Ctrl Pts',(16.2067736327737,-19.3689349046017,-5.81235779956356));
#56829=CARTESIAN_POINT('Ctrl Pts',(16.1944252132089,-19.2855166404035,-5.81654426160515));
#56830=CARTESIAN_POINT('Ctrl Pts',(16.186218055036,-19.2018142528269,-5.82073072364674));
#56831=CARTESIAN_POINT('Ctrl Pts',(16.1780108968631,-19.1181118652502,-5.82491718568833));
#56832=CARTESIAN_POINT('Ctrl Pts',(16.1739449655996,-19.0341258661345,-5.82910364772991));
#56833=CARTESIAN_POINT('Ctrl Pts',(16.1740005630998,-18.9503020392334,-5.8332901097715));
#56834=CARTESIAN_POINT('Ctrl Pts',(16.1712326851452,-18.9503002033939,-5.8332901097715));
#56835=CARTESIAN_POINT('Ctrl Pts',(16.1704460832798,-18.847523176255,-5.83841759033362));
#56836=CARTESIAN_POINT('Ctrl Pts',(16.2227680109981,-17.8958349863275,-5.88593700645621));
#56837=CARTESIAN_POINT('Ctrl Pts',(17.4141948925089,-16.2277744127114,-5.97584835813928));
#56838=CARTESIAN_POINT('Ctrl Pts',(19.4492535155253,-16.3260866525647,-6.06521460822567));
#56839=CARTESIAN_POINT('Ctrl Pts',(20.2230158476471,-16.8629690852954,-6.11218892275159));
#56840=CARTESIAN_POINT('Ctrl Pts',(20.2954006764134,-16.9194747298048,-6.11677130171703));
#56841=CARTESIAN_POINT('',(16.1740007055014,-18.9539005700932,-5.76670989019962));
#56842=CARTESIAN_POINT('Ctrl Pts',(16.174000705501,-18.9539005695105,-5.76670989022851));
#56843=CARTESIAN_POINT('Ctrl Pts',(16.1739381768052,-18.8696766480678,-5.77088500205647));
#56844=CARTESIAN_POINT('Ctrl Pts',(16.1780364138872,-18.7854119279347,-5.77506011388444));
#56845=CARTESIAN_POINT('Ctrl Pts',(16.1862808495761,-18.7015461508315,-5.7792352257124));
#56846=CARTESIAN_POINT('Ctrl Pts',(16.1945245019764,-18.617688341661,-5.78340994087069));
#56847=CARTESIAN_POINT('Ctrl Pts',(16.2069135252697,-18.5342298557721,-5.78758465602899));
#56848=CARTESIAN_POINT('Ctrl Pts',(16.2233814427541,-18.4516056954636,-5.79175937118728));
#56849=CARTESIAN_POINT('Ctrl Pts',(16.2398526754154,-18.3689649019825,-5.79593492676267));
#56850=CARTESIAN_POINT('Ctrl Pts',(16.2604043427349,-18.2871592164315,-5.80011048233807));
#56851=CARTESIAN_POINT('Ctrl Pts',(16.2849190524512,-18.2066125085881,-5.80428603791346));
#56852=CARTESIAN_POINT('Ctrl Pts',(16.3094630809747,-18.1259694694634,-5.80846658731951));
#56853=CARTESIAN_POINT('Ctrl Pts',(16.3379794801119,-18.0465888526479,-5.81264713672555));
#56854=CARTESIAN_POINT('Ctrl Pts',(16.370301376024,-17.9688780263803,-5.8168276861316));
#56855=CARTESIAN_POINT('Ctrl Pts',(16.4026440716432,-17.8911171918327,-5.82101092579452));
#56856=CARTESIAN_POINT('Ctrl Pts',(16.4387969424267,-17.815028700182,-5.82519416545745));
#56857=CARTESIAN_POINT('Ctrl Pts',(16.4785465454209,-17.7409964020585,-5.82937740512037));
#56858=CARTESIAN_POINT('Ctrl Pts',(16.5183679957913,-17.6668302906143,-5.8335682059857));
#56859=CARTESIAN_POINT('Ctrl Pts',(16.5617989238527,-17.5947281861652,-5.83775900685103));
#56860=CARTESIAN_POINT('Ctrl Pts',(16.6085819963934,-17.5250457926251,-5.84194980771636));
#56861=CARTESIAN_POINT('Ctrl Pts',(16.6388616407137,-17.4799449051204,-5.84466224092623));
#56862=CARTESIAN_POINT('Ctrl Pts',(16.67054468148,-17.4358570345709,-5.8473746741361));
#56863=CARTESIAN_POINT('Ctrl Pts',(16.7035527014987,-17.392870830236,-5.85008710734598));
#56864=CARTESIAN_POINT('Ctrl Pts',(16.754476165831,-17.3265534188316,-5.85427174173903));
#56865=CARTESIAN_POINT('Ctrl Pts',(16.8087468503131,-17.262610070515,-5.85845637613208));
#56866=CARTESIAN_POINT('Ctrl Pts',(16.8661152556941,-17.201398222899,-5.86264101052513));
#56867=CARTESIAN_POINT('Ctrl Pts',(16.9234020042507,-17.1402735027716,-5.86681968860906));
#56868=CARTESIAN_POINT('Ctrl Pts',(16.9837774037102,-17.081872893435,-5.870998366693));
#56869=CARTESIAN_POINT('Ctrl Pts',(17.0469505633854,-17.0265223453859,-5.87517704477694));
#56870=CARTESIAN_POINT('Ctrl Pts',(17.1112560565461,-16.9701796785426,-5.87943062266237));
#56871=CARTESIAN_POINT('Ctrl Pts',(17.1784603025299,-16.916997875599,-5.88368420054781));
#56872=CARTESIAN_POINT('Ctrl Pts',(17.248215753932,-16.8672829510612,-5.88793777843324));
#56873=CARTESIAN_POINT('Ctrl Pts',(17.316618859792,-16.8185318473463,-5.8921088924112));
#56874=CARTESIAN_POINT('Ctrl Pts',(17.3874747417493,-16.7731146765033,-5.89628000638915));
#56875=CARTESIAN_POINT('Ctrl Pts',(17.4604222489452,-16.7312794610716,-5.9004511203671));
#56876=CARTESIAN_POINT('Ctrl Pts',(17.5333452779006,-16.6894582838505,-5.90462083468747));
#56877=CARTESIAN_POINT('Ctrl Pts',(17.6083581394473,-16.6512169036016,-5.90879054900784));
#56878=CARTESIAN_POINT('Ctrl Pts',(17.6850725337909,-16.616758862423,-5.91296026332821));
#56879=CARTESIAN_POINT('Ctrl Pts',(17.7617841983071,-16.5823020474093,-5.91712982927226));
#56880=CARTESIAN_POINT('Ctrl Pts',(17.8401968552427,-16.5516284915074,-5.9212993952163));
#56881=CARTESIAN_POINT('Ctrl Pts',(17.9199007999992,-16.5248942147986,-5.92546896116034));
#56882=CARTESIAN_POINT('Ctrl Pts',(18.0024070371279,-16.497219993901,-5.92978512389926));
#56883=CARTESIAN_POINT('Ctrl Pts',(18.0862965548752,-16.4737673840698,-5.93410128663819));
#56884=CARTESIAN_POINT('Ctrl Pts',(18.17109806773,-16.454653124885,-5.93841744937711));
#56885=CARTESIAN_POINT('Ctrl Pts',(18.2531371802229,-16.4361615106827,-5.94259301356879));
#56886=CARTESIAN_POINT('Ctrl Pts',(18.3360293116297,-16.4217299783602,-5.94676857776046));
#56887=CARTESIAN_POINT('Ctrl Pts',(18.4193394847876,-16.4114117295071,-5.95094414195214));
#56888=CARTESIAN_POINT('Ctrl Pts',(18.5068574567408,-16.4005723304336,-5.95533060396469));
#56889=CARTESIAN_POINT('Ctrl Pts',(18.5948362284715,-16.3942727005954,-5.95971706597723));
#56890=CARTESIAN_POINT('Ctrl Pts',(18.6827702698547,-16.3925126461048,-5.96410352798978));
#56891=CARTESIAN_POINT('Ctrl Pts',(18.7707043112378,-16.3907525916143,-5.96848999000232));
#56892=CARTESIAN_POINT('Ctrl Pts',(18.8585930447508,-16.3935320181048,-5.97287645201487));
#56893=CARTESIAN_POINT('Ctrl Pts',(18.9459382820312,-16.4007880988421,-5.97726291402741));
#56894=CARTESIAN_POINT('Ctrl Pts',(19.0292570355294,-16.4077096851946,-5.98144716675294));
#56895=CARTESIAN_POINT('Ctrl Pts',(19.1123913980881,-16.418730040739,-5.98563141947846));
#56896=CARTESIAN_POINT('Ctrl Pts',(19.194905891231,-16.4338328571303,-5.98981567220399));
#56897=CARTESIAN_POINT('Ctrl Pts',(19.2773086561184,-16.4489152236435,-5.99399425926716));
#56898=CARTESIAN_POINT('Ctrl Pts',(19.3590927697209,-16.4680689925776,-5.99817284633033));
#56899=CARTESIAN_POINT('Ctrl Pts',(19.4398267332537,-16.4912260114703,-6.0023514333935));
#56900=CARTESIAN_POINT('Ctrl Pts',(19.5204679325001,-16.5143564226722,-6.00652521921033));
#56901=CARTESIAN_POINT('Ctrl Pts',(19.6000609401166,-16.5414808153857,-6.01069900502716));
#56902=CARTESIAN_POINT('Ctrl Pts',(19.6781847982246,-16.5724800764016,-6.01487279084399));
#56903=CARTESIAN_POINT('Ctrl Pts',(19.756255136842,-16.6034581010796,-6.01904371736923));
#56904=CARTESIAN_POINT('Ctrl Pts',(19.8328578987203,-16.638305552342,-6.02321464389447));
#56905=CARTESIAN_POINT('Ctrl Pts',(19.9075887387112,-16.6768539668034,-6.02738557041971));
#56906=CARTESIAN_POINT('Ctrl Pts',(19.9823054028888,-16.715395068954,-6.03155570575518));
#56907=CARTESIAN_POINT('Ctrl Pts',(20.0551504373947,-16.7576355380431,-6.03572584109066));
#56908=CARTESIAN_POINT('Ctrl Pts',(20.1257419130199,-16.8033598608553,-6.03989597642613));
#56909=CARTESIAN_POINT('Ctrl Pts',(20.1832317946324,-16.8405978684476,-6.04329214550492));
#56910=CARTESIAN_POINT('Ctrl Pts',(20.2392273264478,-16.8801456060531,-6.04668831458371));
#56911=CARTESIAN_POINT('Ctrl Pts',(20.293535888361,-16.9218650751948,-6.05008448366249));
#56912=CARTESIAN_POINT('Ctrl Pts',(20.293535888361,-16.9218650751948,-5.25018234329749));
#56913=CARTESIAN_POINT('Ctrl Pts',(20.3601377623853,-16.9730281833724,-5.25435377502357));
#56914=CARTESIAN_POINT('Ctrl Pts',(20.4242724026374,-17.0275130355736,-5.25852520674965));
#56915=CARTESIAN_POINT('Ctrl Pts',(20.4855962926596,-17.0850478239813,-5.26269663847572));
#56916=CARTESIAN_POINT('Ctrl Pts',(20.5468968472374,-17.1425607188029,-5.2668664828561));
#56917=CARTESIAN_POINT('Ctrl Pts',(20.6053884404635,-17.2031209306373,-5.27103632723647));
#56918=CARTESIAN_POINT('Ctrl Pts',(20.6607620047844,-17.2664175555852,-5.27520617161685));
#56919=CARTESIAN_POINT('Ctrl Pts',(20.716131108673,-17.3297090818852,-5.27937568010935));
#56920=CARTESIAN_POINT('Ctrl Pts',(20.7683823803764,-17.3957362366199,-5.28354518860186));
#56921=CARTESIAN_POINT('Ctrl Pts',(20.817245809119,-17.4641536037655,-5.28771469709437));
#56922=CARTESIAN_POINT('Ctrl Pts',(20.8661199594387,-17.5325859829986,-5.29188512045731));
#56923=CARTESIAN_POINT('Ctrl Pts',(20.9116045244801,-17.6034092410065,-5.29605554382025));
#56924=CARTESIAN_POINT('Ctrl Pts',(20.9534725337246,-17.6762485853261,-5.3002259671832));
#56925=CARTESIAN_POINT('Ctrl Pts',(20.9953878213432,-17.7491701816048,-5.30440109988962));
#56926=CARTESIAN_POINT('Ctrl Pts',(21.033678175198,-17.824112007304,-5.30857623259604));
#56927=CARTESIAN_POINT('Ctrl Pts',(21.0681626420736,-17.9006747599586,-5.31275136530246));
#56928=CARTESIAN_POINT('Ctrl Pts',(21.1026701970053,-17.9772887729425,-5.31692929334565));
#56929=CARTESIAN_POINT('Ctrl Pts',(21.1333666264305,-18.0555254448552,-5.32110722138883));
#56930=CARTESIAN_POINT('Ctrl Pts',(21.1601200340366,-18.1349678216579,-5.32528514943202));
#56931=CARTESIAN_POINT('Ctrl Pts',(21.1869161602422,-18.2145370483607,-5.32946974859679));
#56932=CARTESIAN_POINT('Ctrl Pts',(21.2097565782892,-18.2953153796072,-5.33365434776156));
#56933=CARTESIAN_POINT('Ctrl Pts',(21.228560024071,-18.3768736779567,-5.33783894692634));
#56934=CARTESIAN_POINT('Ctrl Pts',(21.2338697296436,-18.3999040605933,-5.33902059149097));
#56935=CARTESIAN_POINT('Ctrl Pts',(21.2388578513853,-18.4229965973846,-5.34020223605561));
#56936=CARTESIAN_POINT('Ctrl Pts',(21.2435233083642,-18.4461415565825,-5.34138388062024));
#56937=CARTESIAN_POINT('Ctrl Pts',(21.2600453931921,-18.528106298929,-5.34556851501329));
#56938=CARTESIAN_POINT('Ctrl Pts',(21.2725783676242,-18.6110338790214,-5.34975314940634));
#56939=CARTESIAN_POINT('Ctrl Pts',(21.2810167729394,-18.6945013429835,-5.35393778379939));
#56940=CARTESIAN_POINT('Ctrl Pts',(21.2894431672292,-18.7778500013417,-5.35811646188332));
#56941=CARTESIAN_POINT('Ctrl Pts',(21.2937865229904,-18.8617365633854,-5.36229513996726));
#56942=CARTESIAN_POINT('Ctrl Pts',(21.293992315731,-18.9457275683921,-5.3664738180512));
#56943=CARTESIAN_POINT('Ctrl Pts',(21.2942017971586,-19.0312240518004,-5.37072739593664));
#56944=CARTESIAN_POINT('Ctrl Pts',(21.2901238296771,-19.1168282866478,-5.37498097382208));
#56945=CARTESIAN_POINT('Ctrl Pts',(21.2817561480521,-19.202077208203,-5.37923455170751));
#56946=CARTESIAN_POINT('Ctrl Pts',(21.2735506902637,-19.2856734130643,-5.38340566568546));
#56947=CARTESIAN_POINT('Ctrl Pts',(21.2612204100085,-19.3689274796566,-5.38757677966342));
#56948=CARTESIAN_POINT('Ctrl Pts',(21.2448156932502,-19.4514041995501,-5.39174789364137));
#56949=CARTESIAN_POINT('Ctrl Pts',(21.2284164812531,-19.5338532435837,-5.39591760796174));
#56950=CARTESIAN_POINT('Ctrl Pts',(21.2079456377351,-19.6155250081443,-5.40008732228211));
#56951=CARTESIAN_POINT('Ctrl Pts',(21.1835049170499,-19.695993051949,-5.40425703660248));
#56952=CARTESIAN_POINT('Ctrl Pts',(21.1590650660704,-19.7764582323555,-5.40842660254653));
#56953=CARTESIAN_POINT('Ctrl Pts',(21.1306557533066,-19.855719337241,-5.41259616849058));
#56954=CARTESIAN_POINT('Ctrl Pts',(21.0984286192895,-19.9333650209198,-5.41676573443462));
#56955=CARTESIAN_POINT('Ctrl Pts',(21.0650684189968,-20.0137406310503,-5.42108189717355));
#56956=CARTESIAN_POINT('Ctrl Pts',(21.0276171353222,-20.0923846228544,-5.42539805991247));
#56957=CARTESIAN_POINT('Ctrl Pts',(20.9862964849991,-20.1688650474316,-5.42971422265139));
#56958=CARTESIAN_POINT('Ctrl Pts',(20.946321850514,-20.2428541302226,-5.43388978684307));
#56959=CARTESIAN_POINT('Ctrl Pts',(20.9027263517804,-20.314818059135,-5.43806535103475));
#56960=CARTESIAN_POINT('Ctrl Pts',(20.8557557370743,-20.3843940073151,-5.44224091522644));
#56961=CARTESIAN_POINT('Ctrl Pts',(20.8064127482816,-20.4574840712366,-5.44662737723898));
#56962=CARTESIAN_POINT('Ctrl Pts',(20.7533450801509,-20.5279381144881,-5.45101383925152));
#56963=CARTESIAN_POINT('Ctrl Pts',(20.6968850924152,-20.5953752200804,-5.45540030126406));
#56964=CARTESIAN_POINT('Ctrl Pts',(20.6404251046795,-20.6628123256726,-5.4597867632766));
#56965=CARTESIAN_POINT('Ctrl Pts',(20.5805732479923,-20.7272321203106,-5.46417322528913));
#56966=CARTESIAN_POINT('Ctrl Pts',(20.5177042670233,-20.788300380603,-5.46855968730167));
#56967=CARTESIAN_POINT('Ctrl Pts',(20.4577279810629,-20.8465587997145,-5.47274432169472));
#56968=CARTESIAN_POINT('Ctrl Pts',(20.3947828711327,-20.9019841740837,-5.47692895608777));
#56969=CARTESIAN_POINT('Ctrl Pts',(20.3291674917033,-20.9542588927042,-5.48111359048082));
#56970=CARTESIAN_POINT('Ctrl Pts',(20.2636455076449,-21.0064592047331,-5.48529226856476));
#56971=CARTESIAN_POINT('Ctrl Pts',(20.1954611603976,-21.0555174845772,-5.4894709466487));
#56972=CARTESIAN_POINT('Ctrl Pts',(20.124949408759,-21.1011532616994,-5.49364962473264));
#56973=CARTESIAN_POINT('Ctrl Pts',(20.0531737846481,-21.1476070273286,-5.49790320261808));
#56974=CARTESIAN_POINT('Ctrl Pts',(19.9789868438524,-21.1905140507392,-5.50215678050351));
#56975=CARTESIAN_POINT('Ctrl Pts',(19.9027767244008,-21.2296217790711,-5.50641035838895));
#56976=CARTESIAN_POINT('Ctrl Pts',(19.8280440868267,-21.2679713277768,-5.5105814723669));
#56977=CARTESIAN_POINT('Ctrl Pts',(19.7513664452244,-21.3026673605995,-5.51475258634485));
#56978=CARTESIAN_POINT('Ctrl Pts',(19.6731370139766,-21.3335166740922,-5.5189237003228));
#56979=CARTESIAN_POINT('Ctrl Pts',(19.5949338333701,-21.3643556357998,-5.52309341464318));
#56980=CARTESIAN_POINT('Ctrl Pts',(19.5151803248755,-21.3913502731114,-5.52726312896355));
#56981=CARTESIAN_POINT('Ctrl Pts',(19.4342901358277,-21.4143553207574,-5.53143284328392));
#56982=CARTESIAN_POINT('Ctrl Pts',(19.3534028252,-21.4373595497851,-5.53560240922797));
#56983=CARTESIAN_POINT('Ctrl Pts',(19.2713793571593,-21.4563743463907,-5.53977197517202));
#56984=CARTESIAN_POINT('Ctrl Pts',(19.1886476884737,-21.4713045626453,-5.54394154111606));
#56985=CARTESIAN_POINT('Ctrl Pts',(19.1030072763778,-21.486759706885,-5.54825770385498));
#56986=CARTESIAN_POINT('Ctrl Pts',(19.0166084554189,-21.4978376052711,-5.5525738665939));
#56987=CARTESIAN_POINT('Ctrl Pts',(18.9299344373273,-21.5044908807416,-5.55689002933282));
#56988=CARTESIAN_POINT('Ctrl Pts',(18.8460838162585,-21.5109274264636,-5.5610655935245));
#56989=CARTESIAN_POINT('Ctrl Pts',(18.7619761239715,-21.5132232209822,-5.56524115771618));
#56990=CARTESIAN_POINT('Ctrl Pts',(18.6780494593124,-21.511388508413,-5.56941672190786));
#56991=CARTESIAN_POINT('Ctrl Pts',(18.589883858338,-21.5094611288736,-5.5738031839204));
#56992=CARTESIAN_POINT('Ctrl Pts',(18.5019186353064,-21.5029750554617,-5.57818964593294));
#56993=CARTESIAN_POINT('Ctrl Pts',(18.4146539811436,-21.492003566974,-5.58257610794548));
#56994=CARTESIAN_POINT('Ctrl Pts',(18.3273893269809,-21.4810320784863,-5.58696256995802));
#56995=CARTESIAN_POINT('Ctrl Pts',(18.2408257994993,-21.4655753517935,-5.59134903197056));
#56996=CARTESIAN_POINT('Ctrl Pts',(18.1554472698611,-21.4457675790757,-5.59573549398311));
#56997=CARTESIAN_POINT('Ctrl Pts',(18.073997132933,-21.4268711913428,-5.59992012837615));
#56998=CARTESIAN_POINT('Ctrl Pts',(17.9933221701875,-21.4039450190917,-5.60410476276919));
#56999=CARTESIAN_POINT('Ctrl Pts',(17.9138510440903,-21.3770681825714,-5.60828939716223));
#57000=CARTESIAN_POINT('Ctrl Pts',(17.8344930353043,-21.3502296019011,-5.61246807524618));
#57001=CARTESIAN_POINT('Ctrl Pts',(17.7563358916499,-21.3194516726888,-5.61664675333012));
#57002=CARTESIAN_POINT('Ctrl Pts',(17.6797967513075,-21.2848642288925,-5.62082543141407));
#57003=CARTESIAN_POINT('Ctrl Pts',(17.6018857018822,-21.2496568300238,-5.62507900929951));
#57004=CARTESIAN_POINT('Ctrl Pts',(17.5256517013915,-21.2105021111286,-5.62933258718494));
#57005=CARTESIAN_POINT('Ctrl Pts',(17.4515171985767,-21.167589732792,-5.63358616507038));
#57006=CARTESIAN_POINT('Ctrl Pts',(17.3788199377604,-21.1255092946461,-5.63775727904834));
#57007=CARTESIAN_POINT('Ctrl Pts',(17.3081419118298,-21.079815837063,-5.64192839302629));
#57008=CARTESIAN_POINT('Ctrl Pts',(17.2398584137962,-21.0307354137495,-5.64609950700425));
#57009=CARTESIAN_POINT('Ctrl Pts',(17.17159782895,-20.9816714598462,-5.65026922132462));
#57010=CARTESIAN_POINT('Ctrl Pts',(17.1057305494617,-20.9292230656517,-5.65443893564499));
#57011=CARTESIAN_POINT('Ctrl Pts',(17.0426026198914,-20.8736594137781,-5.65860864996536));
#57012=CARTESIAN_POINT('Ctrl Pts',(16.9794769366837,-20.8180977390976,-5.66277821590941));
#57013=CARTESIAN_POINT('Ctrl Pts',(16.9190907543429,-20.759421331729,-5.66694778185345));
#57014=CARTESIAN_POINT('Ctrl Pts',(16.8617557221014,-20.6979385338196,-5.6711173477975));
#57015=CARTESIAN_POINT('Ctrl Pts',(16.8024048608569,-20.6342940765829,-5.67543351053642));
#57016=CARTESIAN_POINT('Ctrl Pts',(16.7463240583277,-20.5676425973537,-5.67974967327534));
#57017=CARTESIAN_POINT('Ctrl Pts',(16.6938147044704,-20.4983647564223,-5.68406583601426));
#57018=CARTESIAN_POINT('Ctrl Pts',(16.643015837292,-20.4313436338724,-5.68824140020594));
#57019=CARTESIAN_POINT('Ctrl Pts',(16.5955595388127,-20.3618650450196,-5.69241696439762));
#57020=CARTESIAN_POINT('Ctrl Pts',(16.5516743299489,-20.2903029066083,-5.6965925285893));
#57021=CARTESIAN_POINT('Ctrl Pts',(16.5055725835126,-20.2151263347087,-5.70097899060184));
#57022=CARTESIAN_POINT('Ctrl Pts',(16.4634124379741,-20.1376507144176,-5.70536545261438));
#57023=CARTESIAN_POINT('Ctrl Pts',(16.4254030213234,-20.0583362915701,-5.70975191462692));
#57024=CARTESIAN_POINT('Ctrl Pts',(16.3873936046726,-19.9790218687225,-5.71413837663946));
#57025=CARTESIAN_POINT('Ctrl Pts',(16.3535350701226,-19.897869208087,-5.718524838652));
#57026=CARTESIAN_POINT('Ctrl Pts',(16.323976493569,-19.8153578044185,-5.72291130066454));
#57027=CARTESIAN_POINT('Ctrl Pts',(16.2911969765866,-19.7238552940422,-5.72777574688618));
#57028=CARTESIAN_POINT('Ctrl Pts',(16.2636032939182,-19.630402505787,-5.73264019310782));
#57029=CARTESIAN_POINT('Ctrl Pts',(16.2413973788046,-19.5355513454785,-5.73750463932946));
#57030=CARTESIAN_POINT('Ctrl Pts',(16.2191773325018,-19.4406398246901,-5.74237218114115));
#57031=CARTESIAN_POINT('Ctrl Pts',(16.2023520711407,-19.3443282665182,-5.74723972295285));
#57032=CARTESIAN_POINT('Ctrl Pts',(16.1910760934491,-19.2471914725933,-5.75210726476454));
#57033=CARTESIAN_POINT('Ctrl Pts',(16.1798001157575,-19.1500546786684,-5.75697480657623));
#57034=CARTESIAN_POINT('Ctrl Pts',(16.1740736044194,-19.0520927805192,-5.76184234838793));
#57035=CARTESIAN_POINT('Ctrl Pts',(16.1740007055014,-18.9539005700933,-5.76670989019962));
#57036=CARTESIAN_POINT('Origin',(18.734,-18.952,1.76670989022851));
#57037=CARTESIAN_POINT('',(20.2961058236219,-16.9185141606304,-4.4501059332472));
#57038=CARTESIAN_POINT('',(20.2910030755688,-16.9251725897442,-4.51667470355372));
#57039=CARTESIAN_POINT('',(20.293535888361,-16.9218650751948,1.76670989022851));
#57040=CARTESIAN_POINT('',(16.1741505039397,-18.9508032548666,-5.03329016024815));
#57041=CARTESIAN_POINT('Ctrl Pts',(20.2910030755688,-16.9251725897442,-4.51667470355372));
#57042=CARTESIAN_POINT('Ctrl Pts',(20.612749297949,-17.1716047206165,-4.53675463058365));
#57043=CARTESIAN_POINT('Ctrl Pts',(21.4403820710291,-18.1629200661967,-4.59922649317405));
#57044=CARTESIAN_POINT('Ctrl Pts',(21.3050298972618,-20.5498409932103,-4.70409029132494));
#57045=CARTESIAN_POINT('Ctrl Pts',(18.7821183084785,-21.9787102934683,-4.83126609800637));
#57046=CARTESIAN_POINT('Ctrl Pts',(16.5671405548292,-20.815635979695,-4.94099937082189));
#57047=CARTESIAN_POINT('Ctrl Pts',(16.1797898378084,-19.4541224957223,-5.00834070807693));
#57048=CARTESIAN_POINT('Ctrl Pts',(16.1776748285763,-18.9508059208577,-5.0332901097715));
#57049=CARTESIAN_POINT('Ctrl Pts',(16.1740002797795,-18.9508031412289,-5.03329016239971));
#57050=CARTESIAN_POINT('Ctrl Pts',(16.1740435234788,-18.8583078019676,-5.03786858507912));
#57051=CARTESIAN_POINT('Ctrl Pts',(16.1791038614083,-18.7659792628304,-5.04244700775854));
#57052=CARTESIAN_POINT('Ctrl Pts',(16.1891023385012,-18.6743385289637,-5.04702543043795));
#57053=CARTESIAN_POINT('Ctrl Pts',(16.1991318881351,-18.5824130006799,-5.05161808160685));
#57054=CARTESIAN_POINT('Ctrl Pts',(16.2141301908472,-18.4911798450087,-5.05621073277575));
#57055=CARTESIAN_POINT('Ctrl Pts',(16.2339673694791,-18.401148979913,-5.06080338394464));
#57056=CARTESIAN_POINT('Ctrl Pts',(16.253896242195,-18.3107019620039,-5.06541726388551));
#57057=CARTESIAN_POINT('Ctrl Pts',(16.2787086950666,-18.2214686541854,-5.07003114382637));
#57058=CARTESIAN_POINT('Ctrl Pts',(16.3082244096464,-18.1339457320907,-5.07464502376723));
#57059=CARTESIAN_POINT('Ctrl Pts',(16.3316224115872,-18.064563657823,-5.07830258630123));
#57060=CARTESIAN_POINT('Ctrl Pts',(16.3579750606108,-17.996256071474,-5.08196014883524));
#57061=CARTESIAN_POINT('Ctrl Pts',(16.3871718743356,-17.9292596866308,-5.08561771136924));
#57062=CARTESIAN_POINT('Ctrl Pts',(16.4205760854036,-17.8526088095457,-5.08980234576229));
#57063=CARTESIAN_POINT('Ctrl Pts',(16.4578017058021,-17.7774535557437,-5.09398698015534));
#57064=CARTESIAN_POINT('Ctrl Pts',(16.4986929228155,-17.7042010295369,-5.09817161454839));
#57065=CARTESIAN_POINT('Ctrl Pts',(16.5395259362428,-17.6310527692343,-5.10235029263233));
#57066=CARTESIAN_POINT('Ctrl Pts',(16.5840139603303,-17.559802255246,-5.10652897071626));
#57067=CARTESIAN_POINT('Ctrl Pts',(16.6319534129312,-17.4908360304906,-5.1107076488002));
#57068=CARTESIAN_POINT('Ctrl Pts',(16.6807521457665,-17.4206336357216,-5.11496122668564));
#57069=CARTESIAN_POINT('Ctrl Pts',(16.7331270652481,-17.3527986694292,-5.11921480457108));
#57070=CARTESIAN_POINT('Ctrl Pts',(16.7888147952352,-17.2877120083459,-5.12346838245651));
#57071=CARTESIAN_POINT('Ctrl Pts',(16.8434229099109,-17.2238871791938,-5.12763949643446));
#57072=CARTESIAN_POINT('Ctrl Pts',(16.9012162179242,-17.1627054093257,-5.13181061041241));
#57073=CARTESIAN_POINT('Ctrl Pts',(16.961904139826,-17.1044945839445,-5.13598172439036));
#57074=CARTESIAN_POINT('Ctrl Pts',(17.0225716973095,-17.046303291768,-5.14015143871074));
#57075=CARTESIAN_POINT('Ctrl Pts',(17.0861316079121,-16.9910812823427,-5.14432115303111));
#57076=CARTESIAN_POINT('Ctrl Pts',(17.1522562065725,-16.9391198316955,-5.14849086735148));
#57077=CARTESIAN_POINT('Ctrl Pts',(17.218378452236,-16.8871602300597,-5.15266043329552));
#57078=CARTESIAN_POINT('Ctrl Pts',(17.2870648422621,-16.838461240085,-5.15682999923957));
#57079=CARTESIAN_POINT('Ctrl Pts',(17.3579554657569,-16.7932731901003,-5.16099956518361));
#57080=CARTESIAN_POINT('Ctrl Pts',(17.4313385161206,-16.7464963840237,-5.16531572792253));
#57081=CARTESIAN_POINT('Ctrl Pts',(17.5070832408524,-16.7034822843461,-5.16963189066145));
#57082=CARTESIAN_POINT('Ctrl Pts',(17.5847604857695,-16.6644579700187,-5.17394805340038));
#57083=CARTESIAN_POINT('Ctrl Pts',(17.6599074026035,-16.6267048686258,-5.17812361759205));
#57084=CARTESIAN_POINT('Ctrl Pts',(17.7368624194977,-16.5926857570979,-5.18229918178373));
#57085=CARTESIAN_POINT('Ctrl Pts',(17.8152162748901,-16.5625572895604,-5.18647474597541));
#57086=CARTESIAN_POINT('Ctrl Pts',(17.8975275972498,-16.5309071047512,-5.19086120798795));
#57087=CARTESIAN_POINT('Ctrl Pts',(17.9813822273943,-16.5035511069692,-5.1952476700005));
#57088=CARTESIAN_POINT('Ctrl Pts',(18.0662895457779,-16.4806111699446,-5.19963413201304));
#57089=CARTESIAN_POINT('Ctrl Pts',(18.1511968641614,-16.4576712329201,-5.20402059402558));
#57090=CARTESIAN_POINT('Ctrl Pts',(18.2371562875636,-16.439147404523,-5.20840705603812));
#57091=CARTESIAN_POINT('Ctrl Pts',(18.3236691980734,-16.4250990060965,-5.21279351805067));
#57092=CARTESIAN_POINT('Ctrl Pts',(18.408989825773,-16.4112442165067,-5.21711952777667));
#57093=CARTESIAN_POINT('Ctrl Pts',(18.4951771225028,-16.4016888928814,-5.22144553750267));
#57094=CARTESIAN_POINT('Ctrl Pts',(18.5817594763928,-16.3965308017955,-5.22577154722868));
#57095=CARTESIAN_POINT('Ctrl Pts',(18.6653746429516,-16.3915494790907,-5.22994930409856));
#57096=CARTESIAN_POINT('Ctrl Pts',(18.7493577227615,-16.3906689763753,-5.23412706096844));
#57097=CARTESIAN_POINT('Ctrl Pts',(18.8332735543601,-16.3939255754758,-5.23830481783833));
#57098=CARTESIAN_POINT('Ctrl Pts',(18.9171071872597,-16.3971789846156,-5.24247848243894));
#57099=CARTESIAN_POINT('Ctrl Pts',(19.0008732457144,-16.4045614313944,-5.24665214703955));
#57100=CARTESIAN_POINT('Ctrl Pts',(19.0841345041026,-16.4160572110087,-5.25082581164016));
#57101=CARTESIAN_POINT('Ctrl Pts',(19.1673391847203,-16.4275451789998,-5.25499664014818));
#57102=CARTESIAN_POINT('Ctrl Pts',(19.2500392922831,-16.4431408649386,-5.2591674686562));
#57103=CARTESIAN_POINT('Ctrl Pts',(19.3318020312623,-16.4627766810873,-5.26333829716423));
#57104=CARTESIAN_POINT('Ctrl Pts',(19.413533738698,-16.4824050448233,-5.26750754271101));
#57105=CARTESIAN_POINT('Ctrl Pts',(19.4943283380498,-16.5060703831817,-5.2716767882578));
#57106=CARTESIAN_POINT('Ctrl Pts',(19.5737638927826,-16.5336541594762,-5.27584603380458));
#57107=CARTESIAN_POINT('Ctrl Pts',(19.6532187797483,-16.561244648835,-5.28001629402076));
#57108=CARTESIAN_POINT('Ctrl Pts',(19.7313135247755,-16.5927553354863,-5.28418655423693));
#57109=CARTESIAN_POINT('Ctrl Pts',(19.8076429176265,-16.6280183121568,-5.2883568144531));
#57110=CARTESIAN_POINT('Ctrl Pts',(19.8839842511284,-16.6632868052199,-5.29252772704734));
#57111=CARTESIAN_POINT('Ctrl Pts',(19.9585592703134,-16.7023085526977,-5.29669863964157));
#57112=CARTESIAN_POINT('Ctrl Pts',(20.0309859639485,-16.7448689641708,-5.3008695522358));
#57113=CARTESIAN_POINT('Ctrl Pts',(20.1034742983524,-16.7874655978756,-5.30504401460217));
#57114=CARTESIAN_POINT('Ctrl Pts',(20.1738102696017,-16.8336066600712,-5.30921847696853));
#57115=CARTESIAN_POINT('Ctrl Pts',(20.2416402523474,-16.8830338645831,-5.31339293933489));
#57116=CARTESIAN_POINT('Ctrl Pts',(20.2591066893483,-16.895761527466,-5.31446787671484));
#57117=CARTESIAN_POINT('Ctrl Pts',(20.2764071271508,-16.9087068769371,-5.31554281409479));
#57118=CARTESIAN_POINT('Ctrl Pts',(20.293535888361,-16.9218650751948,-5.31661775147473));
#57119=CARTESIAN_POINT('',(16.1737368696253,-18.9528355653615,-4.96670989022851));
#57120=CARTESIAN_POINT('Ctrl Pts',(16.1740001363332,-18.952835479442,-4.96670989022851));
#57121=CARTESIAN_POINT('Ctrl Pts',(16.1739730621524,-18.8698772454868,-4.97085977152528));
#57122=CARTESIAN_POINT('Ctrl Pts',(16.1779827035226,-18.7867551328103,-4.97500965282205));
#57123=CARTESIAN_POINT('Ctrl Pts',(16.1860506816107,-18.7038986680416,-4.97915953411883));
#57124=CARTESIAN_POINT('Ctrl Pts',(16.194107496698,-18.6211568449803,-4.98330367356457));
#57125=CARTESIAN_POINT('Ctrl Pts',(16.2062114544436,-18.5386804021303,-4.98744781301032));
#57126=CARTESIAN_POINT('Ctrl Pts',(16.2223321624274,-18.4568993297282,-4.99159195245607));
#57127=CARTESIAN_POINT('Ctrl Pts',(16.2384354396283,-18.3752066844675,-4.99573161098228));
#57128=CARTESIAN_POINT('Ctrl Pts',(16.258546748188,-18.2942083730103,-4.99987126950849));
#57129=CARTESIAN_POINT('Ctrl Pts',(16.2825840079951,-18.2143282341429,-5.0040109280347));
#57130=CARTESIAN_POINT('Ctrl Pts',(16.3066073287289,-18.1344944173239,-5.00814818599595));
#57131=CARTESIAN_POINT('Ctrl Pts',(16.33455194816,-18.0557779336924,-5.0122854439572));
#57132=CARTESIAN_POINT('Ctrl Pts',(16.3662852025775,-17.9785902003439,-5.01642270191845));
#57133=CARTESIAN_POINT('Ctrl Pts',(16.3980099615293,-17.9014231313034,-5.020558852274));
#57134=CARTESIAN_POINT('Ctrl Pts',(16.4335211635118,-17.8257844328042,-5.02469500262956));
#57135=CARTESIAN_POINT('Ctrl Pts',(16.4726375176037,-17.7520667838541,-5.02883115298511));
#57136=CARTESIAN_POINT('Ctrl Pts',(16.5117556109323,-17.6783458571842,-5.03296748724699));
#57137=CARTESIAN_POINT('Ctrl Pts',(16.5544789534253,-17.6065465624547,-5.03710382150887));
#57138=CARTESIAN_POINT('Ctrl Pts',(16.6005803897996,-17.5370368319944,-5.04124015577075));
#57139=CARTESIAN_POINT('Ctrl Pts',(16.646728500548,-17.4674567279532,-5.04538067777228));
#57140=CARTESIAN_POINT('Ctrl Pts',(16.6962612737695,-17.4001712070013,-5.04952119977381));
#57141=CARTESIAN_POINT('Ctrl Pts',(16.7489086678727,-17.3355185113609,-5.05366172177533));
#57142=CARTESIAN_POINT('Ctrl Pts',(16.8015842228024,-17.2708312333184,-5.05780445852127));
#57143=CARTESIAN_POINT('Ctrl Pts',(16.8573774008556,-17.2087799314012,-5.06194719526721));
#57144=CARTESIAN_POINT('Ctrl Pts',(16.9159800655235,-17.1496672011401,-5.06608993201314));
#57145=CARTESIAN_POINT('Ctrl Pts',(16.9746826938398,-17.0904536371675,-5.07023973538449));
#57146=CARTESIAN_POINT('Ctrl Pts',(17.0362040315237,-17.0341889688223,-5.07438953875584));
#57147=CARTESIAN_POINT('Ctrl Pts',(17.1002018437186,-16.9811363353769,-5.07853934212719));
#57148=CARTESIAN_POINT('Ctrl Pts',(17.1438608301676,-16.9449440949669,-5.08137031717058));
#57149=CARTESIAN_POINT('Ctrl Pts',(17.1886716656529,-16.910245843732,-5.08420129221397));
#57150=CARTESIAN_POINT('Ctrl Pts',(17.2345184376715,-16.8771132454428,-5.08703226725736));
#57151=CARTESIAN_POINT('Ctrl Pts',(17.302287307428,-16.8281379601765,-5.09121690165041));
#57152=CARTESIAN_POINT('Ctrl Pts',(17.3725842232475,-16.78239517261,-5.09540153604346));
#57153=CARTESIAN_POINT('Ctrl Pts',(17.4450678487465,-16.7401559934152,-5.09958617043651));
#57154=CARTESIAN_POINT('Ctrl Pts',(17.5174483027761,-16.697976936464,-5.10376484852044));
#57155=CARTESIAN_POINT('Ctrl Pts',(17.5920088899902,-16.6592918118672,-5.10794352660438));
#57156=CARTESIAN_POINT('Ctrl Pts',(17.668377621725,-16.6243297168801,-5.11212220468831));
#57157=CARTESIAN_POINT('Ctrl Pts',(17.7461152080911,-16.5887409514671,-5.11637578257375));
#57158=CARTESIAN_POINT('Ctrl Pts',(17.8257260077699,-16.5570102814917,-5.12062936045919));
#57159=CARTESIAN_POINT('Ctrl Pts',(17.9067894477686,-16.5293314914588,-5.12488293834462));
#57160=CARTESIAN_POINT('Ctrl Pts',(17.9862813148006,-16.5021893087815,-5.12905405232258));
#57161=CARTESIAN_POINT('Ctrl Pts',(18.0671695448446,-16.4789434563412,-5.13322516630053));
#57162=CARTESIAN_POINT('Ctrl Pts',(18.1490371223199,-16.4597282588497,-5.13739628027848));
#57163=CARTESIAN_POINT('Ctrl Pts',(18.230877228339,-16.4405195092033,-5.14156599459885));
#57164=CARTESIAN_POINT('Ctrl Pts',(18.3136955816367,-16.4253388333998,-5.14573570891923));
#57165=CARTESIAN_POINT('Ctrl Pts',(18.3970618790067,-16.4142701675274,-5.1499054232396));
#57166=CARTESIAN_POINT('Ctrl Pts',(18.4804252098461,-16.4032018955256,-5.15407498918365));
#57167=CARTESIAN_POINT('Ctrl Pts',(18.5643359898473,-16.3962454022305,-5.1582445551277));
#57168=CARTESIAN_POINT('Ctrl Pts',(18.6483570024151,-16.3934329641448,-5.16241412107174));
#57169=CARTESIAN_POINT('Ctrl Pts',(18.7353320901336,-16.3905216442056,-5.16673028381067));
#57170=CARTESIAN_POINT('Ctrl Pts',(18.822424779069,-16.3920512290412,-5.17104644654959));
#57171=CARTESIAN_POINT('Ctrl Pts',(18.909150084646,-16.3979987376964,-5.17536260928851));
#57172=CARTESIAN_POINT('Ctrl Pts',(18.9930503225157,-16.4037525068826,-5.17953817348019));
#57173=CARTESIAN_POINT('Ctrl Pts',(19.0766062822588,-16.4136406900189,-5.18371373767187));
#57174=CARTESIAN_POINT('Ctrl Pts',(19.1593859487959,-16.427589812537,-5.18788930186354));
#57175=CARTESIAN_POINT('Ctrl Pts',(19.2463466194998,-16.4422434720726,-5.19227576387609));
#57176=CARTESIAN_POINT('Ctrl Pts',(19.3324499449361,-16.4613789616179,-5.19666222588863));
#57177=CARTESIAN_POINT('Ctrl Pts',(19.4172115835232,-16.4848514572204,-5.20104868790118));
#57178=CARTESIAN_POINT('Ctrl Pts',(19.5019732221104,-16.5083239528229,-5.20543514991372));
#57179=CARTESIAN_POINT('Ctrl Pts',(19.5853926474676,-16.5361331988246,-5.20982161192626));
#57180=CARTESIAN_POINT('Ctrl Pts',(19.6670104728637,-16.5680764572817,-5.21420807393881));
#57181=CARTESIAN_POINT('Ctrl Pts',(19.7448664736167,-16.5985474278376,-5.21839236074251));
#57182=CARTESIAN_POINT('Ctrl Pts',(19.821373063144,-16.6328931302869,-5.22257664754621));
#57183=CARTESIAN_POINT('Ctrl Pts',(19.8961176236036,-16.6709733388428,-5.22676093434992));
#57184=CARTESIAN_POINT('Ctrl Pts',(19.9707478771494,-16.7089953113065,-5.2309388221206));
#57185=CARTESIAN_POINT('Ctrl Pts',(20.0436210503407,-16.7507402336343,-5.23511670989127));
#57186=CARTESIAN_POINT('Ctrl Pts',(20.1143433780762,-16.7960194438258,-5.23929459766195));
#57187=CARTESIAN_POINT('Ctrl Pts',(20.1757784666028,-16.8353525989353,-5.24292384620713));
#57188=CARTESIAN_POINT('Ctrl Pts',(20.2355906143445,-16.877351908466,-5.24655309475231));
#57189=CARTESIAN_POINT('Ctrl Pts',(20.293535888361,-16.9218650751948,-5.25018234329749));
#57190=CARTESIAN_POINT('Ctrl Pts',(20.2961058236222,-16.9185141606307,-4.45010593324722));
#57191=CARTESIAN_POINT('Ctrl Pts',(20.3016500329822,-16.9227661777456,-4.45045503344821));
#57192=CARTESIAN_POINT('Ctrl Pts',(20.9781025678406,-17.4463824914852,-4.49319606920968));
#57193=CARTESIAN_POINT('Ctrl Pts',(21.7484972529808,-19.2278589375158,-4.57832904053163));
#57194=CARTESIAN_POINT('Ctrl Pts',(20.1337364777487,-21.6360323460232,-4.70550484721307));
#57195=CARTESIAN_POINT('Ctrl Pts',(17.2348043616254,-21.581772666889,-4.8326806538945));
#57196=CARTESIAN_POINT('Ctrl Pts',(16.1917618388527,-19.8928505847622,-4.91974900156632));
#57197=CARTESIAN_POINT('Ctrl Pts',(16.1699049957539,-18.998574246681,-4.96442541367765));
#57198=CARTESIAN_POINT('Ctrl Pts',(16.1700997034774,-18.952836752384,-4.96670989022851));
#57199=CARTESIAN_POINT('Origin',(18.734,-18.952,1.76670989022851));
#57200=CARTESIAN_POINT('',(20.293535888361,-16.9218650751948,-3.65004596076623));
#57201=CARTESIAN_POINT('',(20.293535888361,-16.9218650751948,-3.71676815356108));
#57202=CARTESIAN_POINT('',(20.293535888361,-16.9218650751948,1.76670989022851));
#57203=CARTESIAN_POINT('',(16.1740009581142,-18.9542148462772,-4.23329008724971));
#57204=CARTESIAN_POINT('Ctrl Pts',(20.293535888361,-16.9218650751948,-3.71676815356108));
#57205=CARTESIAN_POINT('Ctrl Pts',(20.360101304459,-16.9730001766405,-3.72094076536866));
#57206=CARTESIAN_POINT('Ctrl Pts',(20.4242136557516,-17.0274621982811,-3.72511337717624));
#57207=CARTESIAN_POINT('Ctrl Pts',(20.4855270207266,-17.0849828346625,-3.72928598898382));
#57208=CARTESIAN_POINT('Ctrl Pts',(20.5468084015455,-17.1424734653673,-3.73345642414578));
#57209=CARTESIAN_POINT('Ctrl Pts',(20.6052933602042,-17.203019228744,-3.73762685930775));
#57210=CARTESIAN_POINT('Ctrl Pts',(20.6606699271548,-17.2663123089381,-3.74179729446971));
#57211=CARTESIAN_POINT('Ctrl Pts',(20.716034218668,-17.3295913588252,-3.74596680516274));
#57212=CARTESIAN_POINT('Ctrl Pts',(20.7682911845239,-17.3956161695929,-3.75013631585578));
#57213=CARTESIAN_POINT('Ctrl Pts',(20.8171674786023,-17.4640439334128,-3.75430582654881));
#57214=CARTESIAN_POINT('Ctrl Pts',(20.8660475997594,-17.5324770552174,-3.75847566372006));
#57215=CARTESIAN_POINT('Ctrl Pts',(20.9115462572013,-17.6033131285658,-3.76264550089132));
#57216=CARTESIAN_POINT('Ctrl Pts',(20.9534327836276,-17.6761794330866,-3.76681533806257));
#57217=CARTESIAN_POINT('Ctrl Pts',(20.9953632082252,-17.7491221033938,-3.77098954533186));
#57218=CARTESIAN_POINT('Ctrl Pts',(21.0336737129171,-17.8240988539095,-3.77516375260116));
#57219=CARTESIAN_POINT('Ctrl Pts',(21.0681793259974,-17.9007118025554,-3.77933795987045));
#57220=CARTESIAN_POINT('Ctrl Pts',(21.1027036747927,-17.977366350183,-3.78351443363353));
#57221=CARTESIAN_POINT('Ctrl Pts',(21.133418850014,-18.0556584365516,-3.78769090739661));
#57222=CARTESIAN_POINT('Ctrl Pts',(21.1601887465462,-18.1351718870334,-3.79186738115969));
#57223=CARTESIAN_POINT('Ctrl Pts',(21.1870051419978,-18.214823451218,-3.79605110939672));
#57224=CARTESIAN_POINT('Ctrl Pts',(21.2098624458985,-18.2957001737844,-3.80023483763376));
#57225=CARTESIAN_POINT('Ctrl Pts',(21.2286750199151,-18.3773726903361,-3.80441856587079));
#57226=CARTESIAN_POINT('Ctrl Pts',(21.2428259543193,-18.4388072618799,-3.80756559209883));
#57227=CARTESIAN_POINT('Ctrl Pts',(21.2546893789919,-18.5006918342718,-3.81071261832686));
#57228=CARTESIAN_POINT('Ctrl Pts',(21.2642482087236,-18.5628419315355,-3.8138596445549));
#57229=CARTESIAN_POINT('Ctrl Pts',(21.2769586867287,-18.645483579777,-3.818044278948));
#57230=CARTESIAN_POINT('Ctrl Pts',(21.285639763102,-18.7289023900137,-3.82222891334111));
#57231=CARTESIAN_POINT('Ctrl Pts',(21.2902056694013,-18.8126709803349,-3.82641354773422));
#57232=CARTESIAN_POINT('Ctrl Pts',(21.2947650766981,-18.8963203364363,-3.83059222581822));
#57233=CARTESIAN_POINT('Ctrl Pts',(21.2952209238071,-18.9803180282763,-3.83477090390223));
#57234=CARTESIAN_POINT('Ctrl Pts',(21.2915388082527,-19.0642285359494,-3.83894958198624));
#57235=CARTESIAN_POINT('Ctrl Pts',(21.2877906934233,-19.1496430791655,-3.84320315987166));
#57236=CARTESIAN_POINT('Ctrl Pts',(21.2797547375529,-19.2349668053837,-3.84745673775708));
#57237=CARTESIAN_POINT('Ctrl Pts',(21.2674501116906,-19.3197370413421,-3.8517103156425));
#57238=CARTESIAN_POINT('Ctrl Pts',(21.2553840350109,-19.4028638408624,-3.85588142962051));
#57239=CARTESIAN_POINT('Ctrl Pts',(21.2392133934507,-19.485457943358,-3.86005254359853));
#57240=CARTESIAN_POINT('Ctrl Pts',(21.2190086634415,-19.567086939075,-3.86422365757654));
#57241=CARTESIAN_POINT('Ctrl Pts',(21.1988107133246,-19.6486885433942,-3.86839337189698));
#57242=CARTESIAN_POINT('Ctrl Pts',(21.1745814736227,-19.7293252379224,-3.87256308621741));
#57243=CARTESIAN_POINT('Ctrl Pts',(21.1464423282955,-19.8085757483423,-3.87673280053785));
#57244=CARTESIAN_POINT('Ctrl Pts',(21.1183041842798,-19.8878234386891,-3.88090236648196));
#57245=CARTESIAN_POINT('Ctrl Pts',(21.0862565659974,-19.9656846097694,-3.88507193242607));
#57246=CARTESIAN_POINT('Ctrl Pts',(21.0504699913871,-20.0417553757623,-3.88924149837017));
#57247=CARTESIAN_POINT('Ctrl Pts',(21.0134252049623,-20.1205006960415,-3.89355766110902));
#57248=CARTESIAN_POINT('Ctrl Pts',(20.9723738713786,-20.1973268901843,-3.89787382384787));
#57249=CARTESIAN_POINT('Ctrl Pts',(20.9275574633283,-20.2718127348517,-3.90218998658671));
#57250=CARTESIAN_POINT('Ctrl Pts',(20.884200945055,-20.3438722109659,-3.90636555077845));
#57251=CARTESIAN_POINT('Ctrl Pts',(20.8373211816341,-20.4137411050184,-3.9105411149702));
#57252=CARTESIAN_POINT('Ctrl Pts',(20.7871804520946,-20.4810683539778,-3.91471667916194));
#57253=CARTESIAN_POINT('Ctrl Pts',(20.7345072335068,-20.5517961422236,-3.91910314117434));
#57254=CARTESIAN_POINT('Ctrl Pts',(20.6782353411156,-20.6197183310686,-3.92348960318673));
#57255=CARTESIAN_POINT('Ctrl Pts',(20.6187144099125,-20.684469795716,-3.92787606519913));
#57256=CARTESIAN_POINT('Ctrl Pts',(20.5591934787094,-20.7492212603633,-3.93226252721153));
#57257=CARTESIAN_POINT('Ctrl Pts',(20.4964239761435,-20.8108016487773,-3.93664898922393));
#57258=CARTESIAN_POINT('Ctrl Pts',(20.4307957154099,-20.8688944415817,-3.94103545123633));
#57259=CARTESIAN_POINT('Ctrl Pts',(20.3681871082353,-20.9243142988764,-3.94522008562936));
#57260=CARTESIAN_POINT('Ctrl Pts',(20.3027439921319,-20.9767667301135,-3.94940472002239));
#57261=CARTESIAN_POINT('Ctrl Pts',(20.2347793028206,-21.025948283884,-3.95358935441541));
#57262=CARTESIAN_POINT('Ctrl Pts',(20.1669113528321,-21.0750598338002,-3.95776803249935));
#57263=CARTESIAN_POINT('Ctrl Pts',(20.0965293283134,-21.1209094865297,-3.96194671058328));
#57264=CARTESIAN_POINT('Ctrl Pts',(20.0239808111748,-21.1632325763702,-3.96612538866721));
#57265=CARTESIAN_POINT('Ctrl Pts',(19.9501319140058,-21.2063142771792,-3.97037896655265));
#57266=CARTESIAN_POINT('Ctrl Pts',(19.8740384525298,-21.2457414247198,-3.97463254443809));
#57267=CARTESIAN_POINT('Ctrl Pts',(19.7960998386656,-21.2812797025489,-3.97888612232353));
#57268=CARTESIAN_POINT('Ctrl Pts',(19.7196722169164,-21.3161290015149,-3.98305723630146));
#57269=CARTESIAN_POINT('Ctrl Pts',(19.6414707859433,-21.3472386721819,-3.98722835027939));
#57270=CARTESIAN_POINT('Ctrl Pts',(19.5618972814746,-21.3744339188772,-3.99139946425732));
#57271=CARTESIAN_POINT('Ctrl Pts',(19.4823504786638,-21.4016200399449,-3.99556917857768));
#57272=CARTESIAN_POINT('Ctrl Pts',(19.4014329516939,-21.4248941970684,-3.99973889289803));
#57273=CARTESIAN_POINT('Ctrl Pts',(19.319564628433,-21.4441304271503,-4.00390860721839));
#57274=CARTESIAN_POINT('Ctrl Pts',(19.2376992183983,-21.4633659727245,-4.00807817316242));
#57275=CARTESIAN_POINT('Ctrl Pts',(19.1548835273736,-21.4785637725469,-4.01224773910645));
#57276=CARTESIAN_POINT('Ctrl Pts',(19.0715494575443,-21.4896485894843,-4.01641730505048));
#57277=CARTESIAN_POINT('Ctrl Pts',(18.9852854646228,-21.5011231349107,-4.02073346778942));
#57278=CARTESIAN_POINT('Ctrl Pts',(18.8984664850867,-21.5081900216474,-4.02504963052836));
#57279=CARTESIAN_POINT('Ctrl Pts',(18.8115774056926,-21.5108242898109,-4.0293657932673));
#57280=CARTESIAN_POINT('Ctrl Pts',(18.7275187289215,-21.5133727469659,-4.03354135745896));
#57281=CARTESIAN_POINT('Ctrl Pts',(18.6433949192222,-21.5117729919952,-4.03771692165062));
#57282=CARTESIAN_POINT('Ctrl Pts',(18.5596431317113,-21.5060555362953,-4.04189248584229));
#57283=CARTESIAN_POINT('Ctrl Pts',(18.471661240513,-21.5000493054998,-4.04627894785487));
#57284=CARTESIAN_POINT('Ctrl Pts',(18.3840905205394,-21.4894985417946,-4.05066540986745));
#57285=CARTESIAN_POINT('Ctrl Pts',(18.2974272347522,-21.474499597749,-4.05505187188003));
#57286=CARTESIAN_POINT('Ctrl Pts',(18.210763948965,-21.4595006537034,-4.05943833389261));
#57287=CARTESIAN_POINT('Ctrl Pts',(18.1250086463917,-21.440053731818,-4.06382479590519));
#57288=CARTESIAN_POINT('Ctrl Pts',(18.0406384682269,-21.4163152773655,-4.06821125791777));
#57289=CARTESIAN_POINT('Ctrl Pts',(17.9601502870268,-21.3936690643915,-4.07239589231081));
#57290=CARTESIAN_POINT('Ctrl Pts',(17.8806229756134,-21.3670332665356,-4.07658052670385));
#57291=CARTESIAN_POINT('Ctrl Pts',(17.8024810747699,-21.3365067607239,-4.08076516109689));
#57292=CARTESIAN_POINT('Ctrl Pts',(17.7244503992504,-21.306023705615,-4.08494383918082));
#57293=CARTESIAN_POINT('Ctrl Pts',(17.6478016421986,-21.2716611086066,-4.08912251726475));
#57294=CARTESIAN_POINT('Ctrl Pts',(17.5729454850813,-21.2335679725546,-4.09330119534867));
#57295=CARTESIAN_POINT('Ctrl Pts',(17.4967475851455,-21.1947920444157,-4.09755477323411));
#57296=CARTESIAN_POINT('Ctrl Pts',(17.422407646075,-21.1521506525344,-4.10180835111955));
#57297=CARTESIAN_POINT('Ctrl Pts',(17.3503388850133,-21.1058528080799,-4.10606192900499));
#57298=CARTESIAN_POINT('Ctrl Pts',(17.2796673175155,-21.0604525376831,-4.11023304298293));
#57299=CARTESIAN_POINT('Ctrl Pts',(17.2111800563182,-21.0115365845697,-4.11440415696087));
#57300=CARTESIAN_POINT('Ctrl Pts',(17.1452415288503,-20.959348131329,-4.11857527093882));
#57301=CARTESIAN_POINT('Ctrl Pts',(17.0793251276922,-20.9071771904278,-4.12274498525918));
#57302=CARTESIAN_POINT('Ctrl Pts',(17.01595612214,-20.8517362155439,-4.12691469957954));
#57303=CARTESIAN_POINT('Ctrl Pts',(16.9554677262149,-20.7933101181237,-4.1310844138999));
#57304=CARTESIAN_POINT('Ctrl Pts',(16.8949814827263,-20.7348860997546,-4.13525397984395));
#57305=CARTESIAN_POINT('Ctrl Pts',(16.8373759753517,-20.6734774902646,-4.139423545788));
#57306=CARTESIAN_POINT('Ctrl Pts',(16.7829482470746,-20.6094067266084,-4.14359311173204));
#57307=CARTESIAN_POINT('Ctrl Pts',(16.7266069070151,-20.5430833139417,-4.14790927447097));
#57308=CARTESIAN_POINT('Ctrl Pts',(16.6736713066581,-20.47390746331,-4.1522254372099));
#57309=CARTESIAN_POINT('Ctrl Pts',(16.6244248933205,-20.4022733774286,-4.15654159994883));
#57310=CARTESIAN_POINT('Ctrl Pts',(16.5767826767178,-20.3329727643605,-4.1607171641405));
#57311=CARTESIAN_POINT('Ctrl Pts',(16.5325931948253,-20.2613720362608,-4.16489272833218));
#57312=CARTESIAN_POINT('Ctrl Pts',(16.4920674161606,-20.1878552866412,-4.16906829252386));
#57313=CARTESIAN_POINT('Ctrl Pts',(16.4494947767562,-20.1106253807675,-4.17345475453641));
#57314=CARTESIAN_POINT('Ctrl Pts',(16.4109659295264,-20.0312813353545,-4.17784121654897));
#57315=CARTESIAN_POINT('Ctrl Pts',(16.3766684749372,-19.9502925828358,-4.18222767856152));
#57316=CARTESIAN_POINT('Ctrl Pts',(16.342371020348,-19.8693038303171,-4.18661414057408));
#57317=CARTESIAN_POINT('Ctrl Pts',(16.3123050853067,-19.7866709419478,-4.19100060258663));
#57318=CARTESIAN_POINT('Ctrl Pts',(16.2865973915759,-19.702879798822,-4.19538706459919));
#57319=CARTESIAN_POINT('Ctrl Pts',(16.2566341527394,-19.6052182170345,-4.2004996433589));
#57320=CARTESIAN_POINT('Ctrl Pts',(16.2324986213406,-19.5056900725379,-4.20561222211862));
#57321=CARTESIAN_POINT('Ctrl Pts',(16.2143850329185,-19.404924295726,-4.21072480087833));
#57322=CARTESIAN_POINT('Ctrl Pts',(16.1965183144937,-19.3055318551339,-4.21576770033015));
#57323=CARTESIAN_POINT('Ctrl Pts',(16.1845105456257,-19.2049352741343,-4.22081059978196));
#57324=CARTESIAN_POINT('Ctrl Pts',(16.1785021632643,-19.1037590407164,-4.22585349923378));
#57325=CARTESIAN_POINT('Ctrl Pts',(16.1755487125963,-19.0540253526453,-4.22833236190576));
#57326=CARTESIAN_POINT('Ctrl Pts',(16.174044162412,-19.0041519285503,-4.23081122457773));
#57327=CARTESIAN_POINT('Ctrl Pts',(16.1740009581142,-18.9542148462772,-4.23329008724971));
#57328=CARTESIAN_POINT('Ctrl Pts',(16.1756127776244,-18.9542129983521,-4.2332901097715));
#57329=CARTESIAN_POINT('Ctrl Pts',(16.1805387770827,-18.3551144017957,-4.26304769694121));
#57330=CARTESIAN_POINT('Ctrl Pts',(16.6895187238437,-16.8950156783259,-4.3351972196714));
#57331=CARTESIAN_POINT('Ctrl Pts',(18.6971963271545,-16.1157768135428,-4.42965875093214));
#57332=CARTESIAN_POINT('Ctrl Pts',(19.9334915941914,-16.6513471023293,-4.49436269502317));
#57333=CARTESIAN_POINT('Ctrl Pts',(20.2910030755688,-16.9251725897442,-4.51667470355372));
#57334=CARTESIAN_POINT('',(16.1740010840393,-18.9496440968074,-4.16670989022851));
#57335=CARTESIAN_POINT('Ctrl Pts',(16.174088184599,-18.9496434116999,-4.16670992829755));
#57336=CARTESIAN_POINT('Ctrl Pts',(16.1722334877636,-18.748007243103,-4.17674049236081));
#57337=CARTESIAN_POINT('Ctrl Pts',(16.2862273000593,-17.6962739531831,-4.22916299198455));
#57338=CARTESIAN_POINT('Ctrl Pts',(17.7316712464,-16.0996999541064,-4.32362832696778));
#57339=CARTESIAN_POINT('Ctrl Pts',(19.6284056027312,-16.406435236022,-4.40806309788774));
#57340=CARTESIAN_POINT('Ctrl Pts',(20.2961058236222,-16.9185141606307,-4.45010593324722));
#57341=CARTESIAN_POINT('Ctrl Pts',(20.293535888361,-16.9218650751948,-3.65004596076623));
#57342=CARTESIAN_POINT('Ctrl Pts',(20.3602232257825,-16.9730938357748,-3.65422168175373));
#57343=CARTESIAN_POINT('Ctrl Pts',(20.4243341343203,-17.02757381297,-3.65839740274122));
#57344=CARTESIAN_POINT('Ctrl Pts',(20.485549918636,-17.0850043164147,-3.66257312372872));
#57345=CARTESIAN_POINT('Ctrl Pts',(20.5479163710248,-17.1435143363186,-3.66682733540086));
#57346=CARTESIAN_POINT('Ctrl Pts',(20.6072773997898,-17.2050865762893,-3.67108154707301));
#57347=CARTESIAN_POINT('Ctrl Pts',(20.6633380137791,-17.2693666981226,-3.67533575874516));
#57348=CARTESIAN_POINT('Ctrl Pts',(20.7193986277684,-17.3336468199559,-3.67958997041731));
#57349=CARTESIAN_POINT('Ctrl Pts',(20.7721585715388,-17.4006343914317,-3.68384418208945));
#57350=CARTESIAN_POINT('Ctrl Pts',(20.8213695361432,-17.4699445288447,-3.6880983937616));
#57351=CARTESIAN_POINT('Ctrl Pts',(20.8697756595073,-17.5381211047148,-3.69228302815506));
#57352=CARTESIAN_POINT('Ctrl Pts',(20.914928230553,-17.6087985715452,-3.69646766254852));
#57353=CARTESIAN_POINT('Ctrl Pts',(20.956559006204,-17.6816333348432,-3.70065229694198));
#57354=CARTESIAN_POINT('Ctrl Pts',(20.9981305255987,-17.7543644268708,-3.70483097502633));
#57355=CARTESIAN_POINT('Ctrl Pts',(21.0361899803433,-17.8292463201213,-3.70900965311069));
#57356=CARTESIAN_POINT('Ctrl Pts',(21.0705113959643,-17.905905120685,-3.71318833119505));
#57357=CARTESIAN_POINT('Ctrl Pts',(21.1054479982896,-17.9839379751455,-3.71744190908038));
#57358=CARTESIAN_POINT('Ctrl Pts',(21.1365109555626,-18.0638116724909,-3.72169548696571));
#57359=CARTESIAN_POINT('Ctrl Pts',(21.1635100116305,-18.1451040318682,-3.72594906485105));
#57360=CARTESIAN_POINT('Ctrl Pts',(21.1899856383155,-18.22482038024,-3.73012017882942));
#57361=CARTESIAN_POINT('Ctrl Pts',(21.2125533792703,-18.3059004177639,-3.7342912928078));
#57362=CARTESIAN_POINT('Ctrl Pts',(21.2310824062636,-18.3879260187451,-3.73846240678618));
#57363=CARTESIAN_POINT('Ctrl Pts',(21.249605215663,-18.4699240952438,-3.74263212110699));
#57364=CARTESIAN_POINT('Ctrl Pts',(21.2640919013283,-18.5528666566977,-3.74680183542779));
#57365=CARTESIAN_POINT('Ctrl Pts',(21.2744621331457,-18.6363227121685,-3.75097154974859));
#57366=CARTESIAN_POINT('Ctrl Pts',(21.2848319959458,-18.7197757979147,-3.75514111569307));
#57367=CARTESIAN_POINT('Ctrl Pts',(21.2910856402585,-18.8037418847205,-3.75931068163754));
#57368=CARTESIAN_POINT('Ctrl Pts',(21.293194451632,-18.887783501059,-3.76348024758202));
#57369=CARTESIAN_POINT('Ctrl Pts',(21.2953774062114,-18.9747799169322,-3.76779641032044));
#57370=CARTESIAN_POINT('Ctrl Pts',(21.293118626995,-19.0618567451373,-3.77211257305885));
#57371=CARTESIAN_POINT('Ctrl Pts',(21.2864451550249,-19.148529210526,-3.77642873579727));
#57372=CARTESIAN_POINT('Ctrl Pts',(21.2799890707009,-19.2323783294897,-3.78060429998939));
#57373=CARTESIAN_POINT('Ctrl Pts',(21.2694016000863,-19.3158485639548,-3.78477986418151));
#57374=CARTESIAN_POINT('Ctrl Pts',(21.2547598325397,-19.3985085292069,-3.78895542837363));
#57375=CARTESIAN_POINT('Ctrl Pts',(21.2393785441268,-19.48534345277,-3.7933418903852));
#57376=CARTESIAN_POINT('Ctrl Pts',(21.2195227615801,-19.571283533682,-3.79772835239677));
#57377=CARTESIAN_POINT('Ctrl Pts',(21.1953413592831,-19.6558456599868,-3.80211481440833));
#57378=CARTESIAN_POINT('Ctrl Pts',(21.1711599569862,-19.7404077862916,-3.8065012764199));
#57379=CARTESIAN_POINT('Ctrl Pts',(21.1426531949957,-19.8235914337675,-3.81088773843147));
#57380=CARTESIAN_POINT('Ctrl Pts',(21.1100276507034,-19.9049389293616,-3.81527420044303));
#57381=CARTESIAN_POINT('Ctrl Pts',(21.0789032560606,-19.9825435061126,-3.81945883483597));
#57382=CARTESIAN_POINT('Ctrl Pts',(21.0439149217344,-20.058766045094,-3.8236434692289));
#57383=CARTESIAN_POINT('Ctrl Pts',(21.0052063614282,-20.1331950151471,-3.82782810362184));
#57384=CARTESIAN_POINT('Ctrl Pts',(20.9665528979664,-20.2075180447737,-3.83200678170567));
#57385=CARTESIAN_POINT('Ctrl Pts',(20.9241899370651,-20.2800521717354,-3.8361854597895));
#57386=CARTESIAN_POINT('Ctrl Pts',(20.8783095486357,-20.3504050055795,-3.84036413787333));
#57387=CARTESIAN_POINT('Ctrl Pts',(20.8316067872157,-20.422018863411,-3.84461771575879));
#57388=CARTESIAN_POINT('Ctrl Pts',(20.7812594376514,-20.4913720121106,-3.84887129364426));
#57389=CARTESIAN_POINT('Ctrl Pts',(20.7275195051817,-20.5580759578738,-3.85312487152972));
#57390=CARTESIAN_POINT('Ctrl Pts',(20.6748214261695,-20.6234867174841,-3.85729598550756));
#57391=CARTESIAN_POINT('Ctrl Pts',(20.6188614359627,-20.6863497027061,-3.86146709948541));
#57392=CARTESIAN_POINT('Ctrl Pts',(20.5599202972603,-20.7463285841932,-3.86563821346325));
#57393=CARTESIAN_POINT('Ctrl Pts',(20.5009989368264,-20.8062873391872,-3.8698079277835));
#57394=CARTESIAN_POINT('Ctrl Pts',(20.4390987367875,-20.8633635846449,-3.87397764210375));
#57395=CARTESIAN_POINT('Ctrl Pts',(20.3745386111499,-20.9172564884326,-3.87814735642401));
#57396=CARTESIAN_POINT('Ctrl Pts',(20.3099807828387,-20.9711474744794,-3.88231692236793));
#57397=CARTESIAN_POINT('Ctrl Pts',(20.2427635708238,-21.0218550499287,-3.88648648831186));
#57398=CARTESIAN_POINT('Ctrl Pts',(20.1732393309683,-21.0691183595147,-3.89065605425578));
#57399=CARTESIAN_POINT('Ctrl Pts',(20.1012707046024,-21.118043388763,-3.89497221699484));
#57400=CARTESIAN_POINT('Ctrl Pts',(20.0268302379305,-21.1632771484777,-3.89928837973389));
#57401=CARTESIAN_POINT('Ctrl Pts',(19.9503401869381,-21.2045799763026,-3.90360454247295));
#57402=CARTESIAN_POINT('Ctrl Pts',(19.876341791316,-21.2445373688529,-3.90778010666452));
#57403=CARTESIAN_POINT('Ctrl Pts',(19.8004257365565,-21.280815836347,-3.91195567085608));
#57404=CARTESIAN_POINT('Ctrl Pts',(19.7229964759441,-21.3132466983715,-3.91613123504764));
#57405=CARTESIAN_POINT('Ctrl Pts',(19.6416564474416,-21.3473155661428,-3.92051769706045));
#57406=CARTESIAN_POINT('Ctrl Pts',(19.5586468811864,-21.3771377310941,-3.92490415907325));
#57407=CARTESIAN_POINT('Ctrl Pts',(19.4744545807604,-21.4025768736832,-3.92929062108606));
#57408=CARTESIAN_POINT('Ctrl Pts',(19.3902622803343,-21.4280160162723,-3.93367708309886));
#57409=CARTESIAN_POINT('Ctrl Pts',(19.3048878272885,-21.4490720714144,-3.93806354511167));
#57410=CARTESIAN_POINT('Ctrl Pts',(19.2188278686569,-21.4656710082613,-3.94245000712447));
#57411=CARTESIAN_POINT('Ctrl Pts',(19.1367276562992,-21.4815062034173,-3.94663464151748));
#57412=CARTESIAN_POINT('Ctrl Pts',(19.0536980417282,-21.4933443659488,-3.95081927591048));
#57413=CARTESIAN_POINT('Ctrl Pts',(18.9701628470242,-21.5010835823263,-3.95500391030349));
#57414=CARTESIAN_POINT('Ctrl Pts',(18.8867465543302,-21.5088117828872,-3.9591825883874));
#57415=CARTESIAN_POINT('Ctrl Pts',(18.8028265650696,-21.5124525840588,-3.96336126647131));
#57416=CARTESIAN_POINT('Ctrl Pts',(18.7188367813161,-21.511955092731,-3.96753994455521));
#57417=CARTESIAN_POINT('Ctrl Pts',(18.6333415410503,-21.5114486842286,-3.97179352244066));
#57418=CARTESIAN_POINT('Ctrl Pts',(18.5477744529621,-21.5066540748901,-3.9760471003261));
#57419=CARTESIAN_POINT('Ctrl Pts',(18.4625985845166,-21.4975728769127,-3.98030067821155));
#57420=CARTESIAN_POINT('Ctrl Pts',(18.3790740164893,-21.4886677356787,-3.98447179218945));
#57421=CARTESIAN_POINT('Ctrl Pts',(18.2959261128658,-21.4756407813846,-3.98864290616735));
#57422=CARTESIAN_POINT('Ctrl Pts',(18.2135896449255,-21.4585460423322,-3.99281402014525));
#57423=CARTESIAN_POINT('Ctrl Pts',(18.1312808057821,-21.4414570395846,-3.99698373446557));
#57424=CARTESIAN_POINT('Ctrl Pts',(18.0497833116117,-21.4203030563997,-4.00115344878589));
#57425=CARTESIAN_POINT('Ctrl Pts',(17.9695227367341,-21.3951894142595,-4.00532316310622));
#57426=CARTESIAN_POINT('Ctrl Pts',(17.8892650178723,-21.3700766657704,-4.00949272905021));
#57427=CARTESIAN_POINT('Ctrl Pts',(17.8102445695778,-21.3410046766648,-4.0136622949942));
#57428=CARTESIAN_POINT('Ctrl Pts',(17.7328714533936,-21.3081285264539,-4.0178318609382));
#57429=CARTESIAN_POINT('Ctrl Pts',(17.6527779938924,-21.2740964913578,-4.02214802367717));
#57430=CARTESIAN_POINT('Ctrl Pts',(17.5744503476374,-21.2359880155536,-4.02646418641615));
#57431=CARTESIAN_POINT('Ctrl Pts',(17.498318591899,-21.1940284248139,-4.03078034915512));
#57432=CARTESIAN_POINT('Ctrl Pts',(17.424666820098,-21.1534356633302,-4.03495591334675));
#57433=CARTESIAN_POINT('Ctrl Pts',(17.3530704495471,-21.1092391216314,-4.03913147753838));
#57434=CARTESIAN_POINT('Ctrl Pts',(17.2838902366715,-21.0616875774151,-4.04330704173));
#57435=CARTESIAN_POINT('Ctrl Pts',(17.2112158957012,-21.0117343177416,-4.04769350374265));
#57436=CARTESIAN_POINT('Ctrl Pts',(17.1412086706267,-20.9580785813371,-4.0520799657553));
#57437=CARTESIAN_POINT('Ctrl Pts',(17.074246682156,-20.9010559057928,-4.05646642776795));
#57438=CARTESIAN_POINT('Ctrl Pts',(17.0072846936853,-20.8440332302485,-4.0608528897806));
#57439=CARTESIAN_POINT('Ctrl Pts',(16.9433683113268,-20.7836440693276,-4.06523935179325));
#57440=CARTESIAN_POINT('Ctrl Pts',(16.8828286089282,-20.7202659530956,-4.0696258138059));
#57441=CARTESIAN_POINT('Ctrl Pts',(16.8258191500137,-20.66058359639,-4.07375648865202));
#57442=CARTESIAN_POINT('Ctrl Pts',(16.7715797255597,-20.5980163329693,-4.07788716349815));
#57443=CARTESIAN_POINT('Ctrl Pts',(16.720421868205,-20.5328551822216,-4.08201783834428));
#57444=CARTESIAN_POINT('Ctrl Pts',(16.6693300782615,-20.467778183328,-4.08614317866297));
#57445=CARTESIAN_POINT('Ctrl Pts',(16.6213122506322,-20.4001143092104,-4.09026851898165));
#57446=CARTESIAN_POINT('Ctrl Pts',(16.5766430483355,-20.3301911997632,-4.09439385930034));
#57447=CARTESIAN_POINT('Ctrl Pts',(16.5320173182039,-20.2603361396388,-4.09851518482882));
#57448=CARTESIAN_POINT('Ctrl Pts',(16.4907340001793,-20.1882266026471,-4.1026365103573));
#57449=CARTESIAN_POINT('Ctrl Pts',(16.4530264539488,-20.1142218730582,-4.10675783588578));
#57450=CARTESIAN_POINT('Ctrl Pts',(16.4153436115611,-20.0402656271648,-4.11087646135585));
#57451=CARTESIAN_POINT('Ctrl Pts',(16.3812321043791,-19.9644170734852,-4.11499508682592));
#57452=CARTESIAN_POINT('Ctrl Pts',(16.3508802454214,-19.8870616211443,-4.11911371229599));
#57453=CARTESIAN_POINT('Ctrl Pts',(16.3205285952527,-19.8097067009281,-4.12323230943423));
#57454=CARTESIAN_POINT('Ctrl Pts',(16.2939367323083,-19.7308453355426,-4.12735090657246));
#57455=CARTESIAN_POINT('Ctrl Pts',(16.2712450678812,-19.6508834983921,-4.13146950371069));
#57456=CARTESIAN_POINT('Ctrl Pts',(16.2485547151173,-19.570926283335,-4.1355878627786));
#57457=CARTESIAN_POINT('Ctrl Pts',(16.2297642345971,-19.4898691801182,-4.1397062218465));
#57458=CARTESIAN_POINT('Ctrl Pts',(16.2149637529308,-19.4081319830394,-4.14382458091441));
#57459=CARTESIAN_POINT('Ctrl Pts',(16.2001500672816,-19.3263218655941,-4.14794661410208));
#57460=CARTESIAN_POINT('Ctrl Pts',(16.1893335672674,-19.2438309098088,-4.15206864728976));
#57461=CARTESIAN_POINT('Ctrl Pts',(16.1825528364004,-19.1610869947166,-4.15619068047744));
#57462=CARTESIAN_POINT('Ctrl Pts',(16.1767848147302,-19.0907009692733,-4.1596970837278));
#57463=CARTESIAN_POINT('Ctrl Pts',(16.1739362156169,-19.020132176051,-4.16320348697815));
#57464=CARTESIAN_POINT('Ctrl Pts',(16.1740010840393,-18.9496440968074,-4.16670989022851));
#57465=CARTESIAN_POINT('Origin',(18.734,-18.952,1.76670989022851));
#57466=CARTESIAN_POINT('',(20.2912842963712,-16.9247659399654,-2.85017128767263));
#57467=CARTESIAN_POINT('',(20.293535888361,-16.9218650751948,-2.91665631152786));
#57468=CARTESIAN_POINT('',(20.293535888361,-16.9218650751948,1.76670989022851));
#57469=CARTESIAN_POINT('',(16.1740000028035,-18.9521198080497,-3.43329010980363));
#57470=CARTESIAN_POINT('Ctrl Pts',(20.293535888361,-16.9218650751948,-2.91665631152786));
#57471=CARTESIAN_POINT('Ctrl Pts',(20.3304359427923,-16.950211446889,-2.91898054028019));
#57472=CARTESIAN_POINT('Ctrl Pts',(20.3665290689409,-16.9795381976313,-2.92130476903252));
#57473=CARTESIAN_POINT('Ctrl Pts',(20.401762322946,-17.0097927931959,-2.92362899778485));
#57474=CARTESIAN_POINT('Ctrl Pts',(20.4651976823984,-17.0642643769006,-2.92781363217406));
#57475=CARTESIAN_POINT('Ctrl Pts',(20.5260796023552,-17.1219484370562,-2.93199826656327));
#57476=CARTESIAN_POINT('Ctrl Pts',(20.5840648143939,-17.1825763134451,-2.93618290095248));
#57477=CARTESIAN_POINT('Ctrl Pts',(20.6419674916593,-17.243117893555,-2.94036157903251));
#57478=CARTESIAN_POINT('Ctrl Pts',(20.6969813355446,-17.3065946373119,-2.94454025711253));
#57479=CARTESIAN_POINT('Ctrl Pts',(20.7487967797138,-17.3726982756753,-2.94871893519256));
#57480=CARTESIAN_POINT('Ctrl Pts',(20.8015409785421,-17.439986774327,-2.95297251307897));
#57481=CARTESIAN_POINT('Ctrl Pts',(20.8509706214137,-17.5099969539569,-2.95722609096537));
#57482=CARTESIAN_POINT('Ctrl Pts',(20.8967991444563,-17.5823650629678,-2.96147966885178));
#57483=CARTESIAN_POINT('Ctrl Pts',(20.9417391920986,-17.6533301748853,-2.96565078282566));
#57484=CARTESIAN_POINT('Ctrl Pts',(20.9832162459024,-17.7265621993701,-2.96982189679953));
#57485=CARTESIAN_POINT('Ctrl Pts',(21.0210023907229,-17.801686970939,-2.97399301077341));
#57486=CARTESIAN_POINT('Ctrl Pts',(21.0587758560372,-17.8767865336643,-2.97816272508966));
#57487=CARTESIAN_POINT('Ctrl Pts',(21.0928606655495,-17.953777171463,-2.9823324394059));
#57488=CARTESIAN_POINT('Ctrl Pts',(21.1230748017627,-18.0322600413256,-2.98650215372215));
#57489=CARTESIAN_POINT('Ctrl Pts',(21.153287862827,-18.11074011843,-2.99067171966202));
#57490=CARTESIAN_POINT('Ctrl Pts',(21.1796303599629,-18.190711892398,-2.99484128560189));
#57491=CARTESIAN_POINT('Ctrl Pts',(21.2019688964371,-18.2717577444622,-2.99901085154177));
#57492=CARTESIAN_POINT('Ctrl Pts',(21.2250928283449,-18.3556530688812,-3.00332701428548));
#57493=CARTESIAN_POINT('Ctrl Pts',(21.2439258622492,-18.4406988974017,-3.00764317702919));
#57494=CARTESIAN_POINT('Ctrl Pts',(21.2583771885884,-18.5264182690313,-3.0119593397729));
#57495=CARTESIAN_POINT('Ctrl Pts',(21.2723577644625,-18.6093453409698,-3.01613490396034));
#57496=CARTESIAN_POINT('Ctrl Pts',(21.2822377087348,-18.6929022752308,-3.02031046814777));
#57497=CARTESIAN_POINT('Ctrl Pts',(21.2879876706469,-18.7766518372396,-3.02448603233521));
#57498=CARTESIAN_POINT('Ctrl Pts',(21.2940280494849,-18.8646313908058,-3.02887249435706));
#57499=CARTESIAN_POINT('Ctrl Pts',(21.295510260803,-18.9528229589747,-3.0332589563789));
#57500=CARTESIAN_POINT('Ctrl Pts',(21.2924621252161,-19.0407217776803,-3.03764541840075));
#57501=CARTESIAN_POINT('Ctrl Pts',(21.2894139896292,-19.128620596386,-3.0420318804226));
#57502=CARTESIAN_POINT('Ctrl Pts',(21.2818356329246,-19.2162260941259,-3.04641834244444));
#57503=CARTESIAN_POINT('Ctrl Pts',(21.2698170137414,-19.303044260485,-3.05080480446629));
#57504=CARTESIAN_POINT('Ctrl Pts',(21.2583513890591,-19.3858677941968,-3.05498943886226));
#57505=CARTESIAN_POINT('Ctrl Pts',(21.2428024516836,-19.4682831419495,-3.05917407325824));
#57506=CARTESIAN_POINT('Ctrl Pts',(21.2232102976567,-19.5498562486417,-3.06335870765421));
#57507=CARTESIAN_POINT('Ctrl Pts',(21.2036460306358,-19.6313132461141,-3.06753738574112));
#57508=CARTESIAN_POINT('Ctrl Pts',(21.1800500847572,-19.7119299402854,-3.07171606382802));
#57509=CARTESIAN_POINT('Ctrl Pts',(21.1525141031144,-19.7912791746712,-3.07589474191493));
#57510=CARTESIAN_POINT('Ctrl Pts',(21.1244845588152,-19.8720506869848,-3.08014831979963));
#57511=CARTESIAN_POINT('Ctrl Pts',(21.0923724052599,-19.951508376567,-3.08440189768433));
#57512=CARTESIAN_POINT('Ctrl Pts',(21.0563283883887,-20.0292143967122,-3.08865547556903));
#57513=CARTESIAN_POINT('Ctrl Pts',(21.0209831550867,-20.1054139340948,-3.09282658955003));
#57514=CARTESIAN_POINT('Ctrl Pts',(20.981857354168,-20.1799286784576,-3.09699770353102));
#57515=CARTESIAN_POINT('Ctrl Pts',(20.9391422334474,-20.252364460552,-3.10116881751202));
#57516=CARTESIAN_POINT('Ctrl Pts',(20.8964414461978,-20.3247759361205,-3.10533853183546));
#57517=CARTESIAN_POINT('Ctrl Pts',(20.8501539646467,-20.3951094389618,-3.1095082461589));
#57518=CARTESIAN_POINT('Ctrl Pts',(20.8005166300294,-20.4629960350087,-3.11367796048233));
#57519=CARTESIAN_POINT('Ctrl Pts',(20.7508810617213,-20.5308802153594,-3.11784752642946));
#57520=CARTESIAN_POINT('Ctrl Pts',(20.6978961495658,-20.5963172911853,-3.12201709237659));
#57521=CARTESIAN_POINT('Ctrl Pts',(20.6418408397362,-20.6589690478256,-3.12618665832372));
#57522=CARTESIAN_POINT('Ctrl Pts',(20.5838146944558,-20.7238235628383,-3.13050282105905));
#57523=CARTESIAN_POINT('Ctrl Pts',(20.5224985756086,-20.7856928577379,-3.13481898379438));
#57524=CARTESIAN_POINT('Ctrl Pts',(20.4582443784124,-20.8442424061186,-3.13913514652972));
#57525=CARTESIAN_POINT('Ctrl Pts',(20.3960832548337,-20.9008847092082,-3.1433107107245));
#57526=CARTESIAN_POINT('Ctrl Pts',(20.3311729226015,-20.9544199625776,-3.14748627491928));
#57527=CARTESIAN_POINT('Ctrl Pts',(20.2638651397916,-21.0045868201006,-3.15166183911406));
#57528=CARTESIAN_POINT('Ctrl Pts',(20.1931578010452,-21.0572874862143,-3.15604830111967));
#57529=CARTESIAN_POINT('Ctrl Pts',(20.1198049419666,-21.1062702143003,-3.16043476312528));
#57530=CARTESIAN_POINT('Ctrl Pts',(20.0442460480198,-21.1512851778813,-3.16482122513089));
#57531=CARTESIAN_POINT('Ctrl Pts',(19.968687154073,-21.1963001414623,-3.1692076871365));
#57532=CARTESIAN_POINT('Ctrl Pts',(19.8909227738874,-21.2373471369618,-3.17359414914211));
#57533=CARTESIAN_POINT('Ctrl Pts',(19.8114169849418,-21.2742344068933,-3.17798061114772));
#57534=CARTESIAN_POINT('Ctrl Pts',(19.7355693750926,-21.3094244389056,-3.18216524554016));
#57535=CARTESIAN_POINT('Ctrl Pts',(19.6578547653244,-21.3409601078314,-3.1863498799326));
#57536=CARTESIAN_POINT('Ctrl Pts',(19.578659830513,-21.3686401823022,-3.19053451432504));
#57537=CARTESIAN_POINT('Ctrl Pts',(19.4995776198891,-21.3962808576131,-3.19471319240837));
#57538=CARTESIAN_POINT('Ctrl Pts',(19.4190197000618,-21.4200766888,-3.1988918704917));
#57539=CARTESIAN_POINT('Ctrl Pts',(19.3373948467031,-21.4398735214983,-3.20307054857503));
#57540=CARTESIAN_POINT('Ctrl Pts',(19.2543069264955,-21.4600251981986,-3.20732412646062));
#57541=CARTESIAN_POINT('Ctrl Pts',(19.1701138843276,-21.4760328992744,-3.21157770434621));
#57542=CARTESIAN_POINT('Ctrl Pts',(19.0852654759068,-21.4877863800873,-3.2158312822318));
#57543=CARTESIAN_POINT('Ctrl Pts',(19.0020620194665,-21.4993119967374,-3.22000239620914));
#57544=CARTESIAN_POINT('Ctrl Pts',(18.9182288577839,-21.5067468078097,-3.22417351018648));
#57545=CARTESIAN_POINT('Ctrl Pts',(18.8342009436325,-21.5100382661124,-3.22834462416381));
#57546=CARTESIAN_POINT('Ctrl Pts',(18.7502012258592,-21.5133286199344,-3.23251433848358));
#57547=CARTESIAN_POINT('Ctrl Pts',(18.6660073447033,-21.5124783642369,-3.23668405280334));
#57548=CARTESIAN_POINT('Ctrl Pts',(18.5820577129981,-21.5074869480044,-3.2408537671231));
#57549=CARTESIAN_POINT('Ctrl Pts',(18.4981110685809,-21.5024957093878,-3.24502333306653));
#57550=CARTESIAN_POINT('Ctrl Pts',(18.414409115505,-21.4933636313811,-3.24919289900997));
#57551=CARTESIAN_POINT('Ctrl Pts',(18.3313872270487,-21.4801421943903,-3.2533624649534));
#57552=CARTESIAN_POINT('Ctrl Pts',(18.2454463913858,-21.4664559079809,-3.25767862769305));
#57553=CARTESIAN_POINT('Ctrl Pts',(18.1602348531239,-21.4483874314135,-3.2619947904327));
#57554=CARTESIAN_POINT('Ctrl Pts',(18.0762243702397,-21.4260515800794,-3.26631095317234));
#57555=CARTESIAN_POINT('Ctrl Pts',(17.9949505200244,-21.4044433167599,-3.27048651736342));
#57556=CARTESIAN_POINT('Ctrl Pts',(17.9148011124187,-21.378841616957,-3.2746620815545));
#57557=CARTESIAN_POINT('Ctrl Pts',(17.8361862981299,-21.349400791844,-3.27883764574558));
#57558=CARTESIAN_POINT('Ctrl Pts',(17.7536008364223,-21.3184729806292,-3.28322410775951));
#57559=CARTESIAN_POINT('Ctrl Pts',(17.6727096022459,-21.2833082561226,-3.28761056977344));
#57560=CARTESIAN_POINT('Ctrl Pts',(17.5939605452813,-21.2441409297172,-3.29199703178737));
#57561=CARTESIAN_POINT('Ctrl Pts',(17.5152114883168,-21.2049736033118,-3.2963834938013));
#57562=CARTESIAN_POINT('Ctrl Pts',(17.4386050767024,-21.161804026126,-3.30076995581523));
#57563=CARTESIAN_POINT('Ctrl Pts',(17.364553744478,-21.1149186191895,-3.30515641782916));
#57564=CARTESIAN_POINT('Ctrl Pts',(17.2939096238495,-21.070190479346,-3.30934105222176));
#57565=CARTESIAN_POINT('Ctrl Pts',(17.2253276726157,-21.0219144506012,-3.31352568661436));
#57566=CARTESIAN_POINT('Ctrl Pts',(17.1591863942882,-20.97030674261,-3.31771032100696));
#57567=CARTESIAN_POINT('Ctrl Pts',(17.093139259884,-20.9187724918035,-3.32188899909045));
#57568=CARTESIAN_POINT('Ctrl Pts',(17.0295262575255,-20.8639162618917,-3.32606767717394));
#57569=CARTESIAN_POINT('Ctrl Pts',(16.9686982691563,-20.8059983276908,-3.33024635525743));
#57570=CARTESIAN_POINT('Ctrl Pts',(16.9067799828036,-20.7470422561362,-3.33449993314298));
#57571=CARTESIAN_POINT('Ctrl Pts',(16.8477479425957,-20.6849138964936,-3.33875351102853));
#57572=CARTESIAN_POINT('Ctrl Pts',(16.7919382910611,-20.6199317488055,-3.34300708891408));
#57573=CARTESIAN_POINT('Ctrl Pts',(16.7372106185328,-20.5562094068615,-3.34717820289155));
#57574=CARTESIAN_POINT('Ctrl Pts',(16.6855818186072,-20.4897433069906,-3.35134931686903));
#57575=CARTESIAN_POINT('Ctrl Pts',(16.6373315068437,-20.420870732844,-3.35552043084651));
#57576=CARTESIAN_POINT('Ctrl Pts',(16.5890973859384,-20.352021269555,-3.3596901451664));
#57577=CARTESIAN_POINT('Ctrl Pts',(16.544239765417,-20.2807673121879,-3.36385985948629));
#57578=CARTESIAN_POINT('Ctrl Pts',(16.5029964131481,-20.207477198301,-3.36802957380618));
#57579=CARTESIAN_POINT('Ctrl Pts',(16.4617545284946,-20.1341896923911,-3.37219913974973));
#57580=CARTESIAN_POINT('Ctrl Pts',(16.4241268812486,-20.0588665753509,-3.37636870569329));
#57581=CARTESIAN_POINT('Ctrl Pts',(16.3903058438335,-19.9819017925758,-3.38053827163684));
#57582=CARTESIAN_POINT('Ctrl Pts',(16.3552957004569,-19.9022310229649,-3.38485443437632));
#57583=CARTESIAN_POINT('Ctrl Pts',(16.3243650403573,-19.8208014806367,-3.3891705971158));
#57584=CARTESIAN_POINT('Ctrl Pts',(16.2976726756056,-19.7380719867858,-3.39348675985528));
#57585=CARTESIAN_POINT('Ctrl Pts',(16.2718498118347,-19.6580373975154,-3.39766232404646));
#57586=CARTESIAN_POINT('Ctrl Pts',(16.2499934356292,-19.5767867151056,-3.40183788823764));
#57587=CARTESIAN_POINT('Ctrl Pts',(16.2321958025117,-19.4947483371048,-3.40601345242882));
#57588=CARTESIAN_POINT('Ctrl Pts',(16.2134992532485,-19.4085663956273,-3.41039991444245));
#57589=CARTESIAN_POINT('Ctrl Pts',(16.1992823307861,-19.3215156705806,-3.41478637645608));
#57590=CARTESIAN_POINT('Ctrl Pts',(16.1895904829899,-19.2340996450696,-3.41917283846971));
#57591=CARTESIAN_POINT('Ctrl Pts',(16.1798986351937,-19.1466836195585,-3.42355930048334));
#57592=CARTESIAN_POINT('Ctrl Pts',(16.174731820223,-19.0589028772671,-3.42794576249697));
#57593=CARTESIAN_POINT('Ctrl Pts',(16.1740724460423,-18.9712592442245,-3.43233222451059));
#57594=CARTESIAN_POINT('Ctrl Pts',(16.1740244495167,-18.9648795739235,-3.43265151959756));
#57595=CARTESIAN_POINT('Ctrl Pts',(16.1740003013853,-18.958499723977,-3.43297081468453));
#57596=CARTESIAN_POINT('Ctrl Pts',(16.1740000028035,-18.9521198086917,-3.4332901097715));
#57597=CARTESIAN_POINT('Ctrl Pts',(16.1740000028035,-18.9521198080497,-3.43329010980363));
#57598=CARTESIAN_POINT('Ctrl Pts',(16.173996094898,-18.8686175883754,-3.43746913841141));
#57599=CARTESIAN_POINT('Ctrl Pts',(16.1780820066338,-18.7849577973269,-3.4416481670192));
#57600=CARTESIAN_POINT('Ctrl Pts',(16.1862780259001,-18.7015748760835,-3.44582719562698));
#57601=CARTESIAN_POINT('Ctrl Pts',(16.1944623792895,-18.6183106386623,-3.45000027597724));
#57602=CARTESIAN_POINT('Ctrl Pts',(16.2067451760218,-18.5353229435673,-3.45417335632751));
#57603=CARTESIAN_POINT('Ctrl Pts',(16.2230946976723,-18.4530465324877,-3.45834643667777));
#57604=CARTESIAN_POINT('Ctrl Pts',(16.2396087147061,-18.369942324114,-3.46256150311587));
#57605=CARTESIAN_POINT('Ctrl Pts',(16.2602717621694,-18.2875642714266,-3.46677656955396));
#57606=CARTESIAN_POINT('Ctrl Pts',(16.2849973159137,-18.2063554108437,-3.47099163599205));
#57607=CARTESIAN_POINT('Ctrl Pts',(16.3094325809408,-18.1260999774803,-3.47515721572334));
#57608=CARTESIAN_POINT('Ctrl Pts',(16.3378353258575,-18.0469868800097,-3.47932279545462));
#57609=CARTESIAN_POINT('Ctrl Pts',(16.3700710228284,-17.9694320426107,-3.4834883751859));
#57610=CARTESIAN_POINT('Ctrl Pts',(16.4022960455082,-17.8919028861488,-3.48765257555781));
#57611=CARTESIAN_POINT('Ctrl Pts',(16.4383513227395,-17.8159313907882,-3.49181677592972));
#57612=CARTESIAN_POINT('Ctrl Pts',(16.4780536821042,-17.7419147919373,-3.49598097630164));
#57613=CARTESIAN_POINT('Ctrl Pts',(16.5177548909312,-17.667900338019,-3.50014505599887));
#57614=CARTESIAN_POINT('Ctrl Pts',(16.561102752779,-17.5958410741347,-3.50430913569611));
#57615=CARTESIAN_POINT('Ctrl Pts',(16.6078681568274,-17.5261096166088,-3.50847321539335));
#57616=CARTESIAN_POINT('Ctrl Pts',(16.6556310871524,-17.4548907569615,-3.51272611670991));
#57617=CARTESIAN_POINT('Ctrl Pts',(16.7069587733462,-17.3861005826234,-3.51697901802647));
#57618=CARTESIAN_POINT('Ctrl Pts',(16.7615616490752,-17.320103265583,-3.52123191934302));
#57619=CARTESIAN_POINT('Ctrl Pts',(16.815101261178,-17.255391092332,-3.52540200532769));
#57620=CARTESIAN_POINT('Ctrl Pts',(16.8717892886061,-17.1933642853471,-3.52957209131236));
#57621=CARTESIAN_POINT('Ctrl Pts',(16.9313144499797,-17.134329840772,-3.53374217729703));
#57622=CARTESIAN_POINT('Ctrl Pts',(16.9926128107595,-17.0735368147895,-3.53803648627953));
#57623=CARTESIAN_POINT('Ctrl Pts',(17.0569196193486,-17.0159176096088,-3.54233079526203));
#57624=CARTESIAN_POINT('Ctrl Pts',(17.1238587796064,-16.9617625140729,-3.54662510424453));
#57625=CARTESIAN_POINT('Ctrl Pts',(17.1907979398642,-16.9076074185369,-3.55091941322703));
#57626=CARTESIAN_POINT('Ctrl Pts',(17.2603689845986,-16.8569166856669,-3.55521372220953));
#57627=CARTESIAN_POINT('Ctrl Pts',(17.3321657913458,-16.809930708066,-3.55950803119203));
#57628=CARTESIAN_POINT('Ctrl Pts',(17.4021289421208,-16.7641447297734,-3.56369266558497));
#57629=CARTESIAN_POINT('Ctrl Pts',(17.4744678068902,-16.7217048000894,-3.5678772999779));
#57630=CARTESIAN_POINT('Ctrl Pts',(17.5488288662328,-16.6828659396842,-3.57206193437084));
#57631=CARTESIAN_POINT('Ctrl Pts',(17.6230840818116,-16.6440823615896,-3.57624061245467));
#57632=CARTESIAN_POINT('Ctrl Pts',(17.6993553703909,-16.6088898827214,-3.5804192905385));
#57633=CARTESIAN_POINT('Ctrl Pts',(17.7772605377961,-16.5775001365631,-3.58459796862233));
#57634=CARTESIAN_POINT('Ctrl Pts',(17.8565620993404,-16.5455477517632,-3.58885154650779));
#57635=CARTESIAN_POINT('Ctrl Pts',(17.9375562869753,-16.5175360325719,-3.59310512439325));
#57636=CARTESIAN_POINT('Ctrl Pts',(18.0198140087904,-16.4936390887504,-3.59735870227872));
#57637=CARTESIAN_POINT('Ctrl Pts',(18.1004770041527,-16.4702054338167,-3.60152981625656));
#57638=CARTESIAN_POINT('Ctrl Pts',(18.1823545166279,-16.4507285663625,-3.60570093023439));
#57639=CARTESIAN_POINT('Ctrl Pts',(18.2650237601176,-16.4353233647475,-3.60987204421223));
#57640=CARTESIAN_POINT('Ctrl Pts',(18.3476652631443,-16.4199233324967,-3.61404175853249));
#57641=CARTESIAN_POINT('Ctrl Pts',(18.4310975176832,-16.408592336823,-3.61821147285275));
#57642=CARTESIAN_POINT('Ctrl Pts',(18.5148867965882,-16.4013943064263,-3.622381187173));
#57643=CARTESIAN_POINT('Ctrl Pts',(18.5986730939111,-16.3941965321664,-3.62655075311693));
#57644=CARTESIAN_POINT('Ctrl Pts',(18.6828159319225,-16.3911314692988,-3.63072031906085));
#57645=CARTESIAN_POINT('Ctrl Pts',(18.7668770686618,-16.3922111223079,-3.63488988500478));
#57646=CARTESIAN_POINT('Ctrl Pts',(18.8538936912734,-16.3933287345849,-3.63920604774383));
#57647=CARTESIAN_POINT('Ctrl Pts',(18.9408222331034,-16.398887935209,-3.64352221048289));
#57648=CARTESIAN_POINT('Ctrl Pts',(19.0271792931089,-16.4088433193977,-3.64783837322195));
#57649=CARTESIAN_POINT('Ctrl Pts',(19.110723280963,-16.418474407993,-3.65201393741352));
#57650=CARTESIAN_POINT('Ctrl Pts',(19.1937319902678,-16.4322195436239,-3.65618950160508));
#57651=CARTESIAN_POINT('Ctrl Pts',(19.2757772698984,-16.4499853338117,-3.66036506579665));
#57652=CARTESIAN_POINT('Ctrl Pts',(19.3619664615664,-16.4686484318293,-3.66475152780945));
#57653=CARTESIAN_POINT('Ctrl Pts',(19.4470917766263,-16.4917488722623,-3.66913798982225));
#57654=CARTESIAN_POINT('Ctrl Pts',(19.5306760960808,-16.5191195676866,-3.67352445183505));
#57655=CARTESIAN_POINT('Ctrl Pts',(19.6142604155353,-16.5464902631109,-3.67791091384785));
#57656=CARTESIAN_POINT('Ctrl Pts',(19.6963032254016,-16.578130933778,-3.68229737586066));
#57657=CARTESIAN_POINT('Ctrl Pts',(19.7763550154477,-16.6138177954293,-3.68668383787346));
#57658=CARTESIAN_POINT('Ctrl Pts',(19.8527263004242,-16.6478638983275,-3.69086862549939));
#57659=CARTESIAN_POINT('Ctrl Pts',(19.9275699049938,-16.6857190326234,-3.69505341312532));
#57660=CARTESIAN_POINT('Ctrl Pts',(20.0004799995,-16.7272239638861,-3.69923820075125));
#57661=CARTESIAN_POINT('Ctrl Pts',(20.0732773467746,-16.7686647124574,-3.70341651707547));
#57662=CARTESIAN_POINT('Ctrl Pts',(20.1441467296561,-16.8137438158313,-3.70759483339969));
#57663=CARTESIAN_POINT('Ctrl Pts',(20.2127034231806,-16.8622545163887,-3.71177314972391));
#57664=CARTESIAN_POINT('Ctrl Pts',(20.2400223175747,-16.8815853597736,-3.71343815100296));
#57665=CARTESIAN_POINT('Ctrl Pts',(20.2669742267315,-16.901460586774,-3.71510315228202));
#57666=CARTESIAN_POINT('Ctrl Pts',(20.293535888361,-16.9218650751948,-3.71676815356108));
#57667=CARTESIAN_POINT('',(16.1743944592445,-18.9523823947444,-3.36670986511428));
#57668=CARTESIAN_POINT('Ctrl Pts',(16.1740000284928,-18.9523819467095,-3.3667098902285));
#57669=CARTESIAN_POINT('Ctrl Pts',(16.1739869935966,-18.8650154810558,-3.37103154303558));
#57670=CARTESIAN_POINT('Ctrl Pts',(16.1784506871914,-18.7777135371325,-3.37535319584266));
#57671=CARTESIAN_POINT('Ctrl Pts',(16.1873453738309,-18.6909440385447,-3.37967484864975));
#57672=CARTESIAN_POINT('Ctrl Pts',(16.1966194662204,-18.6004733587883,-3.38418084296216));
#57673=CARTESIAN_POINT('Ctrl Pts',(16.2107109130556,-18.5105820575904,-3.38868683727458));
#57674=CARTESIAN_POINT('Ctrl Pts',(16.2295088315793,-18.4217887333309,-3.39319283158699));
#57675=CARTESIAN_POINT('Ctrl Pts',(16.2475982064586,-18.3363422660913,-3.39752898296558));
#57676=CARTESIAN_POINT('Ctrl Pts',(16.2700454505065,-18.2519128648082,-3.40186513434417));
#57677=CARTESIAN_POINT('Ctrl Pts',(16.296700996459,-18.1689459997304,-3.40620128572276));
#57678=CARTESIAN_POINT('Ctrl Pts',(16.3233900671469,-18.0858747870546,-3.41054289068792));
#57679=CARTESIAN_POINT('Ctrl Pts',(16.3542978445813,-18.0042701592832,-3.41488449565309));
#57680=CARTESIAN_POINT('Ctrl Pts',(16.3892268388776,-17.9245571437398,-3.41922610061825));
#57681=CARTESIAN_POINT('Ctrl Pts',(16.4242296046626,-17.8446757709924,-3.42357687523365));
#57682=CARTESIAN_POINT('Ctrl Pts',(16.4632703651625,-17.7666943545301,-3.42792764984905));
#57683=CARTESIAN_POINT('Ctrl Pts',(16.5061059491331,-17.6910130460184,-3.43227842446446));
#57684=CARTESIAN_POINT('Ctrl Pts',(16.5109248522389,-17.6824990756499,-3.43276787644255));
#57685=CARTESIAN_POINT('Ctrl Pts',(16.515791737601,-17.6740141830169,-3.43325732842064));
#57686=CARTESIAN_POINT('Ctrl Pts',(16.5207062260025,-17.6655589131312,-3.43374678039873));
#57687=CARTESIAN_POINT('Ctrl Pts',(16.5627232942887,-17.5932694654538,-3.43793141479117));
#57688=CARTESIAN_POINT('Ctrl Pts',(16.608363899273,-17.5229061642045,-3.44211604918361));
#57689=CARTESIAN_POINT('Ctrl Pts',(16.6574263400684,-17.4548554395523,-3.44630068357605));
#57690=CARTESIAN_POINT('Ctrl Pts',(16.7064189465521,-17.3869015766835,-3.4504793616594));
#57691=CARTESIAN_POINT('Ctrl Pts',(16.7588234476463,-17.3212541220954,-3.45465803974274));
#57692=CARTESIAN_POINT('Ctrl Pts',(16.8143930615577,-17.2582735752536,-3.45883671782609));
#57693=CARTESIAN_POINT('Ctrl Pts',(16.8709587208714,-17.1941641473616,-3.46309029571167));
#57694=CARTESIAN_POINT('Ctrl Pts',(16.930803836094,-17.1328185931037,-3.46734387359726));
#57695=CARTESIAN_POINT('Ctrl Pts',(16.9936228831504,-17.0745848910946,-3.47159745148285));
#57696=CARTESIAN_POINT('Ctrl Pts',(17.0552240603871,-17.0174801630431,-3.47576856546019));
#57697=CARTESIAN_POINT('Ctrl Pts',(17.1196845346186,-16.9633680324693,-3.47993967943753));
#57698=CARTESIAN_POINT('Ctrl Pts',(17.1866778681087,-16.9125407039709,-3.48411079341487));
#57699=CARTESIAN_POINT('Ctrl Pts',(17.2536487213389,-16.8617304310734,-3.48828050773464));
#57700=CARTESIAN_POINT('Ctrl Pts',(17.3231503796757,-16.8142030489941,-3.49245022205441));
#57701=CARTESIAN_POINT('Ctrl Pts',(17.394823786903,-16.7702101223364,-3.49661993637418));
#57702=CARTESIAN_POINT('Ctrl Pts',(17.4664946436829,-16.726218761136,-3.50078950231762));
#57703=CARTESIAN_POINT('Ctrl Pts',(17.5403367031862,-16.685761845216,-3.50495906826106));
#57704=CARTESIAN_POINT('Ctrl Pts',(17.6159635983351,-16.649046547463,-3.50912863420449));
#57705=CARTESIAN_POINT('Ctrl Pts',(17.694249441846,-16.6110403851223,-3.51344479694413));
#57706=CARTESIAN_POINT('Ctrl Pts',(17.7744474914061,-16.5770440773058,-3.51776095968377));
#57707=CARTESIAN_POINT('Ctrl Pts',(17.8561052781563,-16.5472337208454,-3.52207712242341));
#57708=CARTESIAN_POINT('Ctrl Pts',(17.9351030710676,-16.5183944336202,-3.52625268661449));
#57709=CARTESIAN_POINT('Ctrl Pts',(18.0154664958611,-16.4934726654684,-3.53042825080558));
#57710=CARTESIAN_POINT('Ctrl Pts',(18.0967709615464,-16.4725768508479,-3.53460381499666));
#57711=CARTESIAN_POINT('Ctrl Pts',(18.1821819225493,-16.4506256382959,-3.53899027701058));
#57712=CARTESIAN_POINT('Ctrl Pts',(18.2686309144574,-16.4331178853206,-3.54337673902449));
#57713=CARTESIAN_POINT('Ctrl Pts',(18.3556165397335,-16.4201180997138,-3.54776320103841));
#57714=CARTESIAN_POINT('Ctrl Pts',(18.4426021650097,-16.407118314107,-3.55214966305233));
#57715=CARTESIAN_POINT('Ctrl Pts',(18.5301238388031,-16.3986264761921,-3.55653612506624));
#57716=CARTESIAN_POINT('Ctrl Pts',(18.6176794289204,-16.3946440363642,-3.56092258708016));
#57717=CARTESIAN_POINT('Ctrl Pts',(18.7011876748678,-16.3908456887753,-3.56510628052802));
#57718=CARTESIAN_POINT('Ctrl Pts',(18.7850375342268,-16.3911349078501,-3.56928997397587));
#57719=CARTESIAN_POINT('Ctrl Pts',(18.868795197093,-16.3955512414991,-3.57347366742373));
#57720=CARTESIAN_POINT('Ctrl Pts',(18.9524422754803,-16.3999617443031,-3.57765183717926));
#57721=CARTESIAN_POINT('Ctrl Pts',(19.0359969440168,-16.4084885197953,-3.58183000693479));
#57722=CARTESIAN_POINT('Ctrl Pts',(19.1190226609994,-16.4211192144795,-3.58600817669031));
#57723=CARTESIAN_POINT('Ctrl Pts',(19.2019636761046,-16.4337370234749,-3.59018208392532));
#57724=CARTESIAN_POINT('Ctrl Pts',(19.2843763591288,-16.4504503679969,-3.59435599116033));
#57725=CARTESIAN_POINT('Ctrl Pts',(19.3658279303816,-16.4711949962986,-3.59852989839534));
#57726=CARTESIAN_POINT('Ctrl Pts',(19.4496036347878,-16.4925315503012,-3.60282290359291));
#57727=CARTESIAN_POINT('Ctrl Pts',(19.5323620461702,-16.5181329092784,-3.60711590879049));
#57728=CARTESIAN_POINT('Ctrl Pts',(19.613642592643,-16.5478725264229,-3.61140891398806));
#57729=CARTESIAN_POINT('Ctrl Pts',(19.6925889893505,-16.5767581050134,-3.6155786360938));
#57730=CARTESIAN_POINT('Ctrl Pts',(19.7701408045475,-16.6095472854996,-3.61974835819955));
#57731=CARTESIAN_POINT('Ctrl Pts',(19.8458923492031,-16.6460738511861,-3.62391808030529));
#57732=CARTESIAN_POINT('Ctrl Pts',(19.9250034287628,-16.6842203478312,-3.62827272704878));
#57733=CARTESIAN_POINT('Ctrl Pts',(20.002150345742,-16.7264432362292,-3.63262737379227));
#57734=CARTESIAN_POINT('Ctrl Pts',(20.0768973717721,-16.7724985320291,-3.63698202053576));
#57735=CARTESIAN_POINT('Ctrl Pts',(20.1516443978023,-16.8185538278289,-3.64133666727925));
#57736=CARTESIAN_POINT('Ctrl Pts',(20.2239910606285,-16.8684412099267,-3.64569131402274));
#57737=CARTESIAN_POINT('Ctrl Pts',(20.293535888361,-16.9218650751948,-3.65004596076623));
#57738=CARTESIAN_POINT('Ctrl Pts',(20.2912842963712,-16.9247659399654,-2.85017128767263));
#57739=CARTESIAN_POINT('Ctrl Pts',(20.689119003359,-17.2333456259195,-2.87512870967275));
#57740=CARTESIAN_POINT('Ctrl Pts',(21.5323502495748,-18.3705873153274,-2.94247806723335));
#57741=CARTESIAN_POINT('Ctrl Pts',(21.1037095629711,-20.8355520758667,-3.05221936035442));
#57742=CARTESIAN_POINT('Ctrl Pts',(18.4329096239604,-21.9640817435474,-3.17939516703586));
#57743=CARTESIAN_POINT('Ctrl Pts',(16.4590845454477,-20.6164716802603,-3.28422525531007));
#57744=CARTESIAN_POINT('Ctrl Pts',(16.1776267599649,-19.3569817996596,-3.34666340802382));
#57745=CARTESIAN_POINT('Ctrl Pts',(16.1781627867106,-18.9523866751972,-3.36670962517707));
#57746=CARTESIAN_POINT('Origin',(18.734,-18.952,1.76670989022851));
#57747=CARTESIAN_POINT('',(20.293535888361,-16.9218650751948,-2.05017637630343));
#57748=CARTESIAN_POINT('',(20.293535888361,-16.9218650751948,-2.11663751779963));
#57749=CARTESIAN_POINT('',(20.293535888361,-16.9218650751948,1.76670989022851));
#57750=CARTESIAN_POINT('',(16.1740010149448,-18.9497204131756,-2.63329010980609));
#57751=CARTESIAN_POINT('Ctrl Pts',(20.293535888361,-16.9218650751948,-2.11663751779963));
#57752=CARTESIAN_POINT('Ctrl Pts',(20.3602472256299,-16.9731122722949,-2.12081218273854));
#57753=CARTESIAN_POINT('Ctrl Pts',(20.4243917162535,-17.0276218213591,-2.12498684767744));
#57754=CARTESIAN_POINT('Ctrl Pts',(20.4856474637794,-17.0850958346409,-2.12916151261635));
#57755=CARTESIAN_POINT('Ctrl Pts',(20.5469405643417,-17.1426048949019,-2.13333872321698));
#57756=CARTESIAN_POINT('Ctrl Pts',(20.6053410960536,-17.2030816868678,-2.1375159338176));
#57757=CARTESIAN_POINT('Ctrl Pts',(20.6605654848026,-17.2661929431968,-2.14169314441823));
#57758=CARTESIAN_POINT('Ctrl Pts',(20.7158816143227,-17.3294090422494,-2.14587729435364));
#57759=CARTESIAN_POINT('Ctrl Pts',(20.768010782938,-17.3952679817225,-2.15006144428905));
#57760=CARTESIAN_POINT('Ctrl Pts',(20.8167112396531,-17.4634053969523,-2.15424559422446));
#57761=CARTESIAN_POINT('Ctrl Pts',(20.8412645289459,-17.4977582096496,-2.15635511538172));
#57762=CARTESIAN_POINT('Ctrl Pts',(20.8649469915942,-17.5326897523485,-2.15846463653898));
#57763=CARTESIAN_POINT('Ctrl Pts',(20.8877320902557,-17.5681509896658,-2.16057415769624));
#57764=CARTESIAN_POINT('Ctrl Pts',(20.9329306422981,-17.638495059893,-2.16475879183927));
#57765=CARTESIAN_POINT('Ctrl Pts',(20.9747633711847,-17.7111867434279,-2.16894342598229));
#57766=CARTESIAN_POINT('Ctrl Pts',(21.0129782252709,-17.7858703979656,-2.17312806012532));
#57767=CARTESIAN_POINT('Ctrl Pts',(21.0511386851992,-17.8604477494804,-2.17730673795485));
#57768=CARTESIAN_POINT('Ctrl Pts',(21.0856912912936,-17.9370110341171,-2.18148541578439));
#57769=CARTESIAN_POINT('Ctrl Pts',(21.116427617672,-18.0151762991077,-2.18566409361392));
#57770=CARTESIAN_POINT('Ctrl Pts',(21.1477148729796,-18.0947426263206,-2.18991767156241));
#57771=CARTESIAN_POINT('Ctrl Pts',(21.1750474280233,-18.1759685243987,-2.1941712495109));
#57772=CARTESIAN_POINT('Ctrl Pts',(21.1982547719715,-18.2584234585746,-2.19842482745939));
#57773=CARTESIAN_POINT('Ctrl Pts',(21.2210121944976,-18.33927983665,-2.20259594117397));
#57774=CARTESIAN_POINT('Ctrl Pts',(21.2398027993344,-18.421317558152,-2.20676705488855));
#57775=CARTESIAN_POINT('Ctrl Pts',(21.2545152522161,-18.504112889953,-2.21093816860314));
#57776=CARTESIAN_POINT('Ctrl Pts',(21.2692227681819,-18.5868804389239,-2.21510788265736));
#57777=CARTESIAN_POINT('Ctrl Pts',(21.2798547695695,-18.6704046407403,-2.21927759671159));
#57778=CARTESIAN_POINT('Ctrl Pts',(21.2863509615978,-18.7542512482192,-2.22344731076582));
#57779=CARTESIAN_POINT('Ctrl Pts',(21.2928469224598,-18.838094872027,-2.22761687644128));
#57780=CARTESIAN_POINT('Ctrl Pts',(21.2952073318929,-18.9222604199623,-2.23178644211675));
#57781=CARTESIAN_POINT('Ctrl Pts',(21.2934238553148,-19.0063095649563,-2.23595600779222));
#57782=CARTESIAN_POINT('Ctrl Pts',(21.2915776736488,-19.0933137860529,-2.24027217084101));
#57783=CARTESIAN_POINT('Ctrl Pts',(21.2852907961481,-19.1801927391156,-2.24458833388979));
#57784=CARTESIAN_POINT('Ctrl Pts',(21.2746126736341,-19.2664634200821,-2.24890449693858));
#57785=CARTESIAN_POINT('Ctrl Pts',(21.2642823912523,-19.3499238312634,-2.25308006085834));
#57786=CARTESIAN_POINT('Ctrl Pts',(21.2498426885289,-19.4328145349077,-2.25725562477811));
#57787=CARTESIAN_POINT('Ctrl Pts',(21.2313905396645,-19.514708176939,-2.26143118869787));
#57788=CARTESIAN_POINT('Ctrl Pts',(21.2120064127097,-19.6007380895305,-2.26581765131117));
#57789=CARTESIAN_POINT('Ctrl Pts',(21.1881940056838,-19.6856670076433,-2.27020411392447));
#57790=CARTESIAN_POINT('Ctrl Pts',(21.1601243952761,-19.7690192278313,-2.27459057653778));
#57791=CARTESIAN_POINT('Ctrl Pts',(21.1320547848685,-19.8523714480192,-2.27897703915108));
#57792=CARTESIAN_POINT('Ctrl Pts',(21.0997282551218,-19.9341464586593,-2.28336350176438));
#57793=CARTESIAN_POINT('Ctrl Pts',(21.0633723464422,-20.0138966388639,-2.28774996437768));
#57794=CARTESIAN_POINT('Ctrl Pts',(21.0286892306353,-20.089977387114,-2.29193459890685));
#57795=CARTESIAN_POINT('Ctrl Pts',(20.9902102866637,-20.1644987286812,-2.29611923343602));
#57796=CARTESIAN_POINT('Ctrl Pts',(20.948098122754,-20.2370562255471,-2.30030386796519));
#57797=CARTESIAN_POINT('Ctrl Pts',(20.906045900278,-20.30951044583,-2.30448254618695));
#57798=CARTESIAN_POINT('Ctrl Pts',(20.8603709589155,-20.380005979264,-2.30866122440872));
#57799=CARTESIAN_POINT('Ctrl Pts',(20.8112833253055,-20.4481597462864,-2.31283990263049));
#57800=CARTESIAN_POINT('Ctrl Pts',(20.761315833192,-20.5175351177548,-2.31709348048168));
#57801=CARTESIAN_POINT('Ctrl Pts',(20.7078123007176,-20.5844835062303,-2.32134705833287));
#57802=CARTESIAN_POINT('Ctrl Pts',(20.6510424452111,-20.6486284988939,-2.32560063618407));
#57803=CARTESIAN_POINT('Ctrl Pts',(20.5953731818007,-20.7115299183389,-2.32977175030303));
#57804=CARTESIAN_POINT('Ctrl Pts',(20.5365634319266,-20.7717353099771,-2.33394286442199));
#57805=CARTESIAN_POINT('Ctrl Pts',(20.4749092250507,-20.8289217005868,-2.33811397854095));
#57806=CARTESIAN_POINT('Ctrl Pts',(20.4132757068255,-20.8860889017635,-2.34228369300321));
#57807=CARTESIAN_POINT('Ctrl Pts',(20.3487999642225,-20.940238801272,-2.34645340746548));
#57808=CARTESIAN_POINT('Ctrl Pts',(20.2818144940605,-20.9910856509662,-2.35062312192774));
#57809=CARTESIAN_POINT('Ctrl Pts',(20.2148314075177,-21.0419306913198,-2.35479268801438));
#57810=CARTESIAN_POINT('Ctrl Pts',(20.1453391379196,-21.0894726380872,-2.35896225410102));
#57811=CARTESIAN_POINT('Ctrl Pts',(20.0737017376896,-21.1334672250647,-2.36313182018765));
#57812=CARTESIAN_POINT('Ctrl Pts',(19.999545660235,-21.179008604135,-2.36744798276027));
#57813=CARTESIAN_POINT('Ctrl Pts',(19.9230912497087,-21.2207482563567,-2.3717641453329));
#57814=CARTESIAN_POINT('Ctrl Pts',(19.8447714026877,-21.2584663212307,-2.37608030790552));
#57815=CARTESIAN_POINT('Ctrl Pts',(19.7690028109338,-21.294955726763,-2.38025587224007));
#57816=CARTESIAN_POINT('Ctrl Pts',(19.6914889015738,-21.3276813875219,-2.38443143657462));
#57817=CARTESIAN_POINT('Ctrl Pts',(19.6126415021176,-21.3564935247899,-2.38860700090917));
#57818=CARTESIAN_POINT('Ctrl Pts',(19.5298117168502,-21.3867608913672,-2.39299346260083));
#57819=CARTESIAN_POINT('Ctrl Pts',(19.4455107504569,-21.4127088296375,-2.39737992429249));
#57820=CARTESIAN_POINT('Ctrl Pts',(19.3602311944397,-21.4342236988456,-2.40176638598414));
#57821=CARTESIAN_POINT('Ctrl Pts',(19.2749516384225,-21.4557385680537,-2.4061528476758));
#57822=CARTESIAN_POINT('Ctrl Pts',(19.1886940767213,-21.4728203301028,-2.41053930936746));
#57823=CARTESIAN_POINT('Ctrl Pts',(19.1019580505853,-21.4854180217661,-2.41492577105912));
#57824=CARTESIAN_POINT('Ctrl Pts',(19.0192128717129,-21.4974360758147,-2.41911040544303));
#57825=CARTESIAN_POINT('Ctrl Pts',(18.9357242972402,-21.5054183621376,-2.42329503982695));
#57826=CARTESIAN_POINT('Ctrl Pts',(18.8519204122539,-21.5092826938713,-2.42747967421086));
#57827=CARTESIAN_POINT('Ctrl Pts',(18.7682358117207,-21.5131415252074,-2.4316583522859));
#57828=CARTESIAN_POINT('Ctrl Pts',(18.6842372477568,-21.5128940235269,-2.43583703036095));
#57829=CARTESIAN_POINT('Ctrl Pts',(18.6003605130588,-21.5085094342736,-2.44001570843599));
#57830=CARTESIAN_POINT('Ctrl Pts',(18.5149803479453,-21.5040462543973,-2.44426928632368));
#57831=CARTESIAN_POINT('Ctrl Pts',(18.4297268997696,-21.4952961442209,-2.44852286421137));
#57832=CARTESIAN_POINT('Ctrl Pts',(18.3450626650525,-21.4822821481969,-2.45277644209906));
#57833=CARTESIAN_POINT('Ctrl Pts',(18.2620398119429,-21.4695204539127,-2.45694755606873));
#57834=CARTESIAN_POINT('Ctrl Pts',(18.1795840056911,-21.4526587990536,-2.4611186700384));
#57835=CARTESIAN_POINT('Ctrl Pts',(18.0981270507746,-21.431771278252,-2.46528978400807));
#57836=CARTESIAN_POINT('Ctrl Pts',(18.0166974295212,-21.4108907664585,-2.46945949832042));
#57837=CARTESIAN_POINT('Ctrl Pts',(17.9362664391869,-21.3859871858385,-2.47362921263276));
#57838=CARTESIAN_POINT('Ctrl Pts',(17.857254322942,-21.3571854435283,-2.4777989269451));
#57839=CARTESIAN_POINT('Ctrl Pts',(17.7782450182823,-21.3283847261058,-2.48196849288138));
#57840=CARTESIAN_POINT('Ctrl Pts',(17.7006549192467,-21.2956862811424,-2.48613805881766));
#57841=CARTESIAN_POINT('Ctrl Pts',(17.6248864697078,-21.2592640024329,-2.49030762475394));
#57842=CARTESIAN_POINT('Ctrl Pts',(17.5464540946264,-21.2215611611785,-2.49462378750282));
#57843=CARTESIAN_POINT('Ctrl Pts',(17.4699743261967,-21.1798679825075,-2.49893995025171));
#57844=CARTESIAN_POINT('Ctrl Pts',(17.3958663510849,-21.1344294576552,-2.50325611300059));
#57845=CARTESIAN_POINT('Ctrl Pts',(17.3241724357536,-21.0904710881461,-2.50743167718525));
#57846=CARTESIAN_POINT('Ctrl Pts',(17.2546985266632,-21.0430079392874,-2.51160724136991));
#57847=CARTESIAN_POINT('Ctrl Pts',(17.1877934784102,-20.9923052204494,-2.51578280555457));
#57848=CARTESIAN_POINT('Ctrl Pts',(17.1175092148076,-20.9390416275035,-2.52016926758557));
#57849=CARTESIAN_POINT('Ctrl Pts',(17.0500605848374,-20.8822029788445,-2.52455572961657));
#57850=CARTESIAN_POINT('Ctrl Pts',(16.9858097729218,-20.8221419544912,-2.52894219164756));
#57851=CARTESIAN_POINT('Ctrl Pts',(16.9215589610062,-20.762080930138,-2.53332865367856));
#57852=CARTESIAN_POINT('Ctrl Pts',(16.8605063152545,-20.698798000471,-2.53771511570956));
#57853=CARTESIAN_POINT('Ctrl Pts',(16.802965079949,-20.6326856153201,-2.54210157774055));
#57854=CARTESIAN_POINT('Ctrl Pts',(16.7485317522925,-20.5701440813406,-2.54625111891253));
#57855=CARTESIAN_POINT('Ctrl Pts',(16.6970294692199,-20.5048282635504,-2.5504006600845));
#57856=CARTESIAN_POINT('Ctrl Pts',(16.6487573722081,-20.4370465256145,-2.55455020125647));
#57857=CARTESIAN_POINT('Ctrl Pts',(16.6005493742832,-20.3693547930394,-2.55869423237572));
#57858=CARTESIAN_POINT('Ctrl Pts',(16.5555633203296,-20.2992040148308,-2.56283826349496));
#57859=CARTESIAN_POINT('Ctrl Pts',(16.514059720175,-20.2269373137572,-2.5669822946142));
#57860=CARTESIAN_POINT('Ctrl Pts',(16.4725982721948,-20.154744008692,-2.5711221169438));
#57861=CARTESIAN_POINT('Ctrl Pts',(16.4346124893252,-20.0804394498693,-2.57526193927339));
#57862=CARTESIAN_POINT('Ctrl Pts',(16.4003201033268,-20.0043963796323,-2.57940176160299));
#57863=CARTESIAN_POINT('Ctrl Pts',(16.3660518421397,-19.9284068059566,-2.58353867155335));
#57864=CARTESIAN_POINT('Ctrl Pts',(16.3354720095443,-19.8506815753093,-2.58767558150371));
#57865=CARTESIAN_POINT('Ctrl Pts',(16.3087521158423,-19.7716174109842,-2.59181249145407));
#57866=CARTESIAN_POINT('Ctrl Pts',(16.2820372325143,-19.6925680723558,-2.59594862567282));
#57867=CARTESIAN_POINT('Ctrl Pts',(16.2591810094483,-19.6121807387927,-2.60008475989157));
#57868=CARTESIAN_POINT('Ctrl Pts',(16.2403061251851,-19.5308703297896,-2.60422089411032));
#57869=CARTESIAN_POINT('Ctrl Pts',(16.2214331728165,-19.4495682431231,-2.60835660498473));
#57870=CARTESIAN_POINT('Ctrl Pts',(16.2065408484312,-19.3673437264668,-2.61249231585914));
#57871=CARTESIAN_POINT('Ctrl Pts',(16.1957010120584,-19.2846232821293,-2.61662802673355));
#57872=CARTESIAN_POINT('Ctrl Pts',(16.1848552750847,-19.2018578094073,-2.62076598885772));
#57873=CARTESIAN_POINT('Ctrl Pts',(16.1780664813587,-19.1185963356398,-2.62490395098188));
#57874=CARTESIAN_POINT('Ctrl Pts',(16.1753546619781,-19.0352708485527,-2.62904191310604));
#57875=CARTESIAN_POINT('Ctrl Pts',(16.1744266413966,-19.0067557610314,-2.63045797866119));
#57876=CARTESIAN_POINT('Ctrl Pts',(16.1739756253558,-18.9782331861948,-2.63187404421635));
#57877=CARTESIAN_POINT('Ctrl Pts',(16.1740010149441,-18.949720413872,-2.6332901097715));
#57878=CARTESIAN_POINT('Ctrl Pts',(16.1740010149447,-18.9497204131756,-2.63329010980609));
#57879=CARTESIAN_POINT('Ctrl Pts',(16.1740928743929,-18.8465613267996,-2.63841342883191));
#57880=CARTESIAN_POINT('Ctrl Pts',(16.1804238944876,-18.7436786900648,-2.64353674785773));
#57881=CARTESIAN_POINT('Ctrl Pts',(16.1928719236877,-18.6417289897893,-2.64866006688355));
#57882=CARTESIAN_POINT('Ctrl Pts',(16.2055250386107,-18.5380996318225,-2.6538677944185));
#57883=CARTESIAN_POINT('Ctrl Pts',(16.2244983314994,-18.4354341185118,-2.65907552195346));
#57884=CARTESIAN_POINT('Ctrl Pts',(16.249614957165,-18.3343990293583,-2.66428324948841));
#57885=CARTESIAN_POINT('Ctrl Pts',(16.2576437833537,-18.3021019692125,-2.66594796113293));
#57886=CARTESIAN_POINT('Ctrl Pts',(16.2662999939976,-18.2699713447297,-2.66761267277746));
#57887=CARTESIAN_POINT('Ctrl Pts',(16.2755767948953,-18.2380284707337,-2.66927738442199));
#57888=CARTESIAN_POINT('Ctrl Pts',(16.2988961609904,-18.1577327328976,-2.67346201883521));
#57889=CARTESIAN_POINT('Ctrl Pts',(16.3261969265523,-18.0784312369418,-2.67764665324844));
#57890=CARTESIAN_POINT('Ctrl Pts',(16.3573766633345,-18.0005476808496,-2.68183128766167));
#57891=CARTESIAN_POINT('Ctrl Pts',(16.3885120196229,-17.9227749823538,-2.68600996576607));
#57892=CARTESIAN_POINT('Ctrl Pts',(16.4235152107073,-17.8464166382457,-2.69018864387046));
#57893=CARTESIAN_POINT('Ctrl Pts',(16.4622338002164,-17.7718820679608,-2.69436732197485));
#57894=CARTESIAN_POINT('Ctrl Pts',(16.5016463923759,-17.6960115195324,-2.69862089985521));
#57895=CARTESIAN_POINT('Ctrl Pts',(16.5449087556002,-17.6220312333017,-2.70287447773556));
#57896=CARTESIAN_POINT('Ctrl Pts',(16.5918084260802,-17.55035266182,-2.70712805561592));
#57897=CARTESIAN_POINT('Ctrl Pts',(16.6377988552168,-17.4800637188785,-2.71129916961483));
#57898=CARTESIAN_POINT('Ctrl Pts',(16.6872865541291,-17.4119884433508,-2.71547028361375));
#57899=CARTESIAN_POINT('Ctrl Pts',(16.7400252973108,-17.3464892136658,-2.71964139761266));
#57900=CARTESIAN_POINT('Ctrl Pts',(16.7927463434997,-17.2810119628776,-2.72381111195414));
#57901=CARTESIAN_POINT('Ctrl Pts',(16.8487159791043,-17.2181093992061,-2.72798082629562));
#57902=CARTESIAN_POINT('Ctrl Pts',(16.9076465125814,-17.1581123393607,-2.7321505406371));
#57903=CARTESIAN_POINT('Ctrl Pts',(16.9665749490588,-17.0981174144665,-2.73632010660236));
#57904=CARTESIAN_POINT('Ctrl Pts',(17.0284637509529,-17.0410281154314,-2.74048967256763));
#57905=CARTESIAN_POINT('Ctrl Pts',(17.0929880053966,-16.987138774985,-2.7446592385329));
#57906=CARTESIAN_POINT('Ctrl Pts',(17.1597808523048,-16.9313547524114,-2.74897540124711));
#57907=CARTESIAN_POINT('Ctrl Pts',(17.2293975200619,-16.8790002342604,-2.75329156396132));
#57908=CARTESIAN_POINT('Ctrl Pts',(17.3014414464083,-16.8303553571507,-2.75760772667553));
#57909=CARTESIAN_POINT('Ctrl Pts',(17.3711385501861,-16.7832950812868,-2.76178329088851));
#57910=CARTESIAN_POINT('Ctrl Pts',(17.4431067778018,-16.7397066785438,-2.76595885510149));
#57911=CARTESIAN_POINT('Ctrl Pts',(17.5169602827153,-16.6997978939377,-2.77013441931447));
#57912=CARTESIAN_POINT('Ctrl Pts',(17.5945439513522,-16.6578734121651,-2.7745208812793));
#57913=CARTESIAN_POINT('Ctrl Pts',(17.6742078257199,-16.6200102829154,-2.77890734324412));
#57914=CARTESIAN_POINT('Ctrl Pts',(17.7554809190364,-16.5863921694013,-2.78329380520895));
#57915=CARTESIAN_POINT('Ctrl Pts',(17.8367540123529,-16.5527740558871,-2.78768026717377));
#57916=CARTESIAN_POINT('Ctrl Pts',(17.9196357523207,-16.523401080228,-2.79206672913859));
#57917=CARTESIAN_POINT('Ctrl Pts',(18.0036392138267,-16.4983958913426,-2.79645319110342));
#57918=CARTESIAN_POINT('Ctrl Pts',(18.0837805456623,-16.4745403370102,-2.80063798179662));
#57919=CARTESIAN_POINT('Ctrl Pts',(18.1652410320983,-16.4545709643755,-2.80482277248982));
#57920=CARTESIAN_POINT('Ctrl Pts',(18.2476089212221,-16.4386310023227,-2.80900756318302));
#57921=CARTESIAN_POINT('Ctrl Pts',(18.3298587386536,-16.4227138896876,-2.81318635511476));
#57922=CARTESIAN_POINT('Ctrl Pts',(18.4130129271248,-16.4108148007751,-2.8173651470465));
#57923=CARTESIAN_POINT('Ctrl Pts',(18.4966446832037,-16.4030271767654,-2.82154393897824));
#57924=CARTESIAN_POINT('Ctrl Pts',(18.5801762046828,-16.3952488864037,-2.82571772253091));
#57925=CARTESIAN_POINT('Ctrl Pts',(18.6641837002162,-16.3915723068656,-2.82989150608357));
#57926=CARTESIAN_POINT('Ctrl Pts',(18.748231717209,-16.392039559246,-2.83406528963623));
#57927=CARTESIAN_POINT('Ctrl Pts',(18.8322246249333,-16.3925065052547,-2.83823633648948));
#57928=CARTESIAN_POINT('Ctrl Pts',(18.9162575426882,-16.3971118856053,-2.84240738334274));
#57929=CARTESIAN_POINT('Ctrl Pts',(18.999892508799,-16.4058458071506,-2.84657843019599));
#57930=CARTESIAN_POINT('Ctrl Pts',(19.083497725474,-16.41457662199,-2.85074799338403));
#57931=CARTESIAN_POINT('Ctrl Pts',(19.1667048146443,-16.4274330128491,-2.85491755657206));
#57932=CARTESIAN_POINT('Ctrl Pts',(19.2490798028144,-16.4443531355606,-2.8590871197601));
#57933=CARTESIAN_POINT('Ctrl Pts',(19.3314501999323,-16.4612723152533,-2.86325645056349));
#57934=CARTESIAN_POINT('Ctrl Pts',(19.4129881380691,-16.4822546823773,-2.86742578136688));
#57935=CARTESIAN_POINT('Ctrl Pts',(19.4932700684874,-16.5071873357864,-2.87159511217027));
#57936=CARTESIAN_POINT('Ctrl Pts',(19.5736163334742,-16.5321399691772,-2.87576778410031));
#57937=CARTESIAN_POINT('Ctrl Pts',(19.6527041405874,-16.5610490742656,-2.87994045603036));
#57938=CARTESIAN_POINT('Ctrl Pts',(19.7301259599796,-16.5937521182338,-2.8841131279604));
#57939=CARTESIAN_POINT('Ctrl Pts',(19.80758106589,-16.6264692224563,-2.88828759387722));
#57940=CARTESIAN_POINT('Ctrl Pts',(19.8833683419596,-16.6629833163712,-2.89246205979404));
#57941=CARTESIAN_POINT('Ctrl Pts',(19.957103132272,-16.7030849887498,-2.89663652571085));
#57942=CARTESIAN_POINT('Ctrl Pts',(20.0309449059727,-16.7432448455048,-2.90081704844978));
#57943=CARTESIAN_POINT('Ctrl Pts',(20.1027278532674,-16.7870024370963,-2.90499757118871));
#57944=CARTESIAN_POINT('Ctrl Pts',(20.1720950490366,-16.8341041975733,-2.90917809392763));
#57945=CARTESIAN_POINT('Ctrl Pts',(20.213456940573,-16.8621897773121,-2.91167083312771));
#57946=CARTESIAN_POINT('Ctrl Pts',(20.2539605186504,-16.891463544437,-2.91416357232779));
#57947=CARTESIAN_POINT('Ctrl Pts',(20.293535888361,-16.9218650751948,-2.91665631152786));
#57948=CARTESIAN_POINT('',(16.1740009418753,-18.9541959965583,-2.56670989022851));
#57949=CARTESIAN_POINT('Ctrl Pts',(16.172685086933,-18.9541844540912,-2.56671052146184));
#57950=CARTESIAN_POINT('Ctrl Pts',(16.1790130664392,-18.2584131946872,-2.60137099441126));
#57951=CARTESIAN_POINT('Ctrl Pts',(16.8320815170599,-16.7012241087188,-2.67842340292117));
#57952=CARTESIAN_POINT('Ctrl Pts',(18.9167593652634,-16.1584579179283,-2.77291032499143));
#57953=CARTESIAN_POINT('Ctrl Pts',(20.0133687891635,-16.7092013388142,-2.83273677411227));
#57954=CARTESIAN_POINT('Ctrl Pts',(20.2912842963712,-16.9247659399654,-2.85017128767263));
#57955=CARTESIAN_POINT('Ctrl Pts',(20.293535888361,-16.9218650751948,-2.05017637630343));
#57956=CARTESIAN_POINT('Ctrl Pts',(20.3599947739675,-16.972918340639,-2.05435390936659));
#57957=CARTESIAN_POINT('Ctrl Pts',(20.424037310397,-17.0273100671775,-2.05853144242976));
#57958=CARTESIAN_POINT('Ctrl Pts',(20.4853117242371,-17.0847808793423,-2.06270897549293));
#57959=CARTESIAN_POINT('Ctrl Pts',(20.5465213916427,-17.1421909641996,-2.06688209430953));
#57960=CARTESIAN_POINT('Ctrl Pts',(20.6049684159709,-17.2026733548758,-2.07105521312614));
#57961=CARTESIAN_POINT('Ctrl Pts',(20.6603338894341,-17.2659283092295,-2.07522833194274));
#57962=CARTESIAN_POINT('Ctrl Pts',(20.7156675790622,-17.3291469506085,-2.07939905508363));
#57963=CARTESIAN_POINT('Ctrl Pts',(20.7679229277693,-17.3951346502392,-2.08356977822452));
#57964=CARTESIAN_POINT('Ctrl Pts',(20.8168185234436,-17.4635555104741,-2.08774050136541));
#57965=CARTESIAN_POINT('Ctrl Pts',(20.8657007171828,-17.5319576170377,-2.09191008134074));
#57966=CARTESIAN_POINT('Ctrl Pts',(20.9112247197038,-17.6027911854591,-2.09607966131607));
#57967=CARTESIAN_POINT('Ctrl Pts',(20.9531508455286,-17.6756890955611,-2.1002492412914));
#57968=CARTESIAN_POINT('Ctrl Pts',(20.9950780564932,-17.7485888924203,-2.10441892918458));
#57969=CARTESIAN_POINT('Ctrl Pts',(21.0334069776191,-17.8235527376139,-2.10858861707775));
#57970=CARTESIAN_POINT('Ctrl Pts',(21.0679432156334,-17.9001877229283,-2.11275830497093));
#57971=CARTESIAN_POINT('Ctrl Pts',(21.1025145462378,-17.9769005777583,-2.11693222972244));
#57972=CARTESIAN_POINT('Ctrl Pts',(21.1332853065668,-18.0552875441195,-2.12110615447396));
#57973=CARTESIAN_POINT('Ctrl Pts',(21.1601089504552,-18.1349349104745,-2.12528007922547));
#57974=CARTESIAN_POINT('Ctrl Pts',(21.1869458980825,-18.2146217795823,-2.12945607412099));
#57975=CARTESIAN_POINT('Ctrl Pts',(21.2098317045075,-18.2955698507065,-2.13363206901651));
#57976=CARTESIAN_POINT('Ctrl Pts',(21.2286701992247,-18.3773517622928,-2.13780806391203));
#57977=CARTESIAN_POINT('Ctrl Pts',(21.2475424633262,-18.4592802739571,-2.14199154458485));
#57978=CARTESIAN_POINT('Ctrl Pts',(21.2623528380693,-18.5420451588483,-2.14617502525768));
#57979=CARTESIAN_POINT('Ctrl Pts',(21.273056640464,-18.6252105012155,-2.15035850593051));
#57980=CARTESIAN_POINT('Ctrl Pts',(21.2829756094017,-18.7022779224197,-2.15423524181513));
#57981=CARTESIAN_POINT('Ctrl Pts',(21.2893686864234,-18.7796888801639,-2.15811197769975));
#57982=CARTESIAN_POINT('Ctrl Pts',(21.2922402934534,-18.8570968865022,-2.16198871358438));
#57983=CARTESIAN_POINT('Ctrl Pts',(21.2953399702062,-18.9406528171088,-2.16617334886797));
#57984=CARTESIAN_POINT('Ctrl Pts',(21.2943475192283,-19.0245162609818,-2.17035798415156));
#57985=CARTESIAN_POINT('Ctrl Pts',(21.2892270081162,-19.1082527983545,-2.17454261943515));
#57986=CARTESIAN_POINT('Ctrl Pts',(21.2841137854036,-19.1918701473637,-2.17872129842001));
#57987=CARTESIAN_POINT('Ctrl Pts',(21.274884201526,-19.2753604934237,-2.18289997740487));
#57988=CARTESIAN_POINT('Ctrl Pts',(21.2615542857184,-19.3582872539799,-2.18707865638973));
#57989=CARTESIAN_POINT('Ctrl Pts',(21.2479854443897,-19.4427003944775,-2.19133223405123));
#57990=CARTESIAN_POINT('Ctrl Pts',(21.2301678127852,-19.5265290647065,-2.19558581171274));
#57991=CARTESIAN_POINT('Ctrl Pts',(21.208173766456,-19.6093158855382,-2.19983938937424));
#57992=CARTESIAN_POINT('Ctrl Pts',(21.1866061117414,-19.6904977444785,-2.20401050427198));
#57993=CARTESIAN_POINT('Ctrl Pts',(21.1610226544758,-19.7706773244638,-2.20818161916971));
#57994=CARTESIAN_POINT('Ctrl Pts',(21.1315432451786,-19.8494332217488,-2.21235273406745));
#57995=CARTESIAN_POINT('Ctrl Pts',(21.1020737279442,-19.9281626918327,-2.21652244931264));
#57996=CARTESIAN_POINT('Ctrl Pts',(21.0687110161701,-20.0054689975125,-2.22069216455782));
#57997=CARTESIAN_POINT('Ctrl Pts',(21.0316242449842,-20.0809476643586,-2.22486187980301));
#57998=CARTESIAN_POINT('Ctrl Pts',(20.9945387934706,-20.1564236454194,-2.22903144667569));
#57999=CARTESIAN_POINT('Ctrl Pts',(20.9537297496554,-20.2300717044421,-2.23320101354836));
#58000=CARTESIAN_POINT('Ctrl Pts',(20.9094130507601,-20.3015103032518,-2.23737058042103));
#58001=CARTESIAN_POINT('Ctrl Pts',(20.8635382531532,-20.3754605600038,-2.24168674207477));
#58002=CARTESIAN_POINT('Ctrl Pts',(20.8139048344501,-20.4470426505681,-2.2460029037285));
#58003=CARTESIAN_POINT('Ctrl Pts',(20.7608012117367,-20.515865994292,-2.25031906538223));
#58004=CARTESIAN_POINT('Ctrl Pts',(20.7094274096053,-20.582447456381,-2.25449463050257));
#58005=CARTESIAN_POINT('Ctrl Pts',(20.6548063539525,-20.6464468137819,-2.2586701956229));
#58006=CARTESIAN_POINT('Ctrl Pts',(20.5972390425424,-20.7075455762656,-2.26284576074324));
#58007=CARTESIAN_POINT('Ctrl Pts',(20.5367641853794,-20.7717302471062,-2.26723222066367));
#58008=CARTESIAN_POINT('Ctrl Pts',(20.4730380462215,-20.8327132050707,-2.2716186805841));
#58009=CARTESIAN_POINT('Ctrl Pts',(20.4064500165861,-20.8901720620268,-2.27600514050453));
#58010=CARTESIAN_POINT('Ctrl Pts',(20.3398619869507,-20.9476309189828,-2.28039160042496));
#58011=CARTESIAN_POINT('Ctrl Pts',(20.2704125717478,-21.0015653791251,-2.28477806034539));
#58012=CARTESIAN_POINT('Ctrl Pts',(20.1985254700657,-21.0517059669222,-2.28916452026582));
#58013=CARTESIAN_POINT('Ctrl Pts',(20.1299459675163,-21.0995395349505,-2.29334915467529));
#58014=CARTESIAN_POINT('Ctrl Pts',(20.0588929044663,-21.1440987240594,-2.29753378908477));
#58015=CARTESIAN_POINT('Ctrl Pts',(19.9857121094434,-21.1851181775877,-2.30171842349424));
#58016=CARTESIAN_POINT('Ctrl Pts',(19.9126354781746,-21.226079245029,-2.30589710159743));
#58017=CARTESIAN_POINT('Ctrl Pts',(19.8374375284691,-21.2635103616748,-2.31007577970061));
#58018=CARTESIAN_POINT('Ctrl Pts',(19.7604940332823,-21.2971886916911,-2.3142544578038));
#58019=CARTESIAN_POINT('Ctrl Pts',(19.6821713816853,-21.3314706813749,-2.31850803568478));
#58020=CARTESIAN_POINT('Ctrl Pts',(19.6020403867589,-21.3618637479467,-2.32276161356576));
#58021=CARTESIAN_POINT('Ctrl Pts',(19.5205248076212,-21.3881811769646,-2.32701519144673));
#58022=CARTESIAN_POINT('Ctrl Pts',(19.4405895664662,-21.413988391455,-2.33118630545076));
#58023=CARTESIAN_POINT('Ctrl Pts',(19.3593234056757,-21.4358764386427,-2.33535741945479));
#58024=CARTESIAN_POINT('Ctrl Pts',(19.2771455317525,-21.4537179959654,-2.33952853345882));
#58025=CARTESIAN_POINT('Ctrl Pts',(19.194995233359,-21.4715535663921,-2.34369824780777));
#58026=CARTESIAN_POINT('Ctrl Pts',(19.1119342786071,-21.485345246116,-2.34786796215672));
#58027=CARTESIAN_POINT('Ctrl Pts',(19.0283943159569,-21.4950163166469,-2.35203767650567));
#58028=CARTESIAN_POINT('Ctrl Pts',(18.9448573259675,-21.5046870430453,-2.35620724248077));
#58029=CARTESIAN_POINT('Ctrl Pts',(18.8608418190481,-21.5102373997256,-2.36037680845588));
#58030=CARTESIAN_POINT('Ctrl Pts',(18.7767854909901,-21.5116424363103,-2.36454637443098));
#58031=CARTESIAN_POINT('Ctrl Pts',(18.6897738473697,-21.5130968722274,-2.36886253714067));
#58032=CARTESIAN_POINT('Ctrl Pts',(18.6027189860106,-21.5101090568378,-2.37317869985036));
#58033=CARTESIAN_POINT('Ctrl Pts',(18.5161054386262,-21.5027100893915,-2.37749486256005));
#58034=CARTESIAN_POINT('Ctrl Pts',(18.4323133171285,-21.4955521424197,-2.3816704267887));
#58035=CARTESIAN_POINT('Ctrl Pts',(18.3489346599974,-21.4842661264524,-2.38584599101735));
#58036=CARTESIAN_POINT('Ctrl Pts',(18.266400191337,-21.4689327402492,-2.390021555246));
#58037=CARTESIAN_POINT('Ctrl Pts',(18.1796971048713,-21.452824901532,-2.39440801719621));
#58038=CARTESIAN_POINT('Ctrl Pts',(18.0939262957253,-21.4322502184638,-2.39879447914641));
#58039=CARTESIAN_POINT('Ctrl Pts',(18.0095696123222,-21.4073616054278,-2.40318094109662));
#58040=CARTESIAN_POINT('Ctrl Pts',(17.9252129289191,-21.3824729923918,-2.40756740304683));
#58041=CARTESIAN_POINT('Ctrl Pts',(17.8422708932844,-21.3532707138249,-2.41195386499704));
#58042=CARTESIAN_POINT('Ctrl Pts',(17.7611994326681,-21.3199651720832,-2.41634032694725));
#58043=CARTESIAN_POINT('Ctrl Pts',(17.6838581936353,-21.288192069127,-2.42052496109126));
#58044=CARTESIAN_POINT('Ctrl Pts',(17.6079312972239,-21.2525667345156,-2.42470959523527));
#58045=CARTESIAN_POINT('Ctrl Pts',(17.5338290567893,-21.2132363226944,-2.42889422937928));
#58046=CARTESIAN_POINT('Ctrl Pts',(17.4598322918057,-21.1739618928909,-2.4330729072098));
#58047=CARTESIAN_POINT('Ctrl Pts',(17.3876554268637,-21.1309930749775,-2.43725158504032));
#58048=CARTESIAN_POINT('Ctrl Pts',(17.3176892303927,-21.0845252176456,-2.44143026287085));
#58049=CARTESIAN_POINT('Ctrl Pts',(17.246468934763,-21.0372244537998,-2.44568384081909));
#58050=CARTESIAN_POINT('Ctrl Pts',(17.1775397859107,-20.9862981588104,-2.44993741876734));
#58051=CARTESIAN_POINT('Ctrl Pts',(17.1112881539936,-20.9320015820273,-2.45419099671558));
#58052=CARTESIAN_POINT('Ctrl Pts',(17.046320944286,-20.8787576544711,-2.4583621104312));
#58053=CARTESIAN_POINT('Ctrl Pts',(16.983928731977,-20.8222732634782,-2.46253322414681));
#58054=CARTESIAN_POINT('Ctrl Pts',(16.9244454837175,-20.762831978015,-2.46670433786243));
#58055=CARTESIAN_POINT('Ctrl Pts',(16.8649821956771,-20.7034106386898,-2.4708740519177));
#58056=CARTESIAN_POINT('Ctrl Pts',(16.8084262582069,-20.641034700359,-2.47504376597298));
#58057=CARTESIAN_POINT('Ctrl Pts',(16.7550758225426,-20.5760255847352,-2.47921348002825));
#58058=CARTESIAN_POINT('Ctrl Pts',(16.7017272853469,-20.5110187824527,-2.48338304570478));
#58059=CARTESIAN_POINT('Ctrl Pts',(16.651584314341,-20.4433793453335,-2.4875526113813));
#58060=CARTESIAN_POINT('Ctrl Pts',(16.6049048052798,-20.3734618010412,-2.49172217705783));
#58061=CARTESIAN_POINT('Ctrl Pts',(16.5565840957098,-20.3010860323251,-2.4960383401054));
#58062=CARTESIAN_POINT('Ctrl Pts',(16.5119752240842,-20.2262694173157,-2.50035450315297));
#58063=CARTESIAN_POINT('Ctrl Pts',(16.4713143087945,-20.1494362040685,-2.50467066620054));
#58064=CARTESIAN_POINT('Ctrl Pts',(16.4319779239082,-20.0751058347982,-2.50884623012138));
#58065=CARTESIAN_POINT('Ctrl Pts',(16.3963363916713,-19.9988886782757,-2.51302179404221));
#58066=CARTESIAN_POINT('Ctrl Pts',(16.3645549999889,-19.9211905859647,-2.51719735796305));
#58067=CARTESIAN_POINT('Ctrl Pts',(16.3311683990456,-19.8395681312915,-2.52158382057399));
#58068=CARTESIAN_POINT('Ctrl Pts',(16.3020423326888,-19.7563117555003,-2.52597028318493));
#58069=CARTESIAN_POINT('Ctrl Pts',(16.2773090396202,-19.6719093867897,-2.53035674579587));
#58070=CARTESIAN_POINT('Ctrl Pts',(16.2525757465516,-19.5875070180792,-2.53474320840681));
#58071=CARTESIAN_POINT('Ctrl Pts',(16.2322352869843,-19.5019592385255,-2.53912967101775));
#58072=CARTESIAN_POINT('Ctrl Pts',(16.2163575306375,-19.4157632978817,-2.54351613362869));
#58073=CARTESIAN_POINT('Ctrl Pts',(16.193544110504,-19.2919155599045,-2.54981867488562));
#58074=CARTESIAN_POINT('Ctrl Pts',(16.1798641823048,-19.1663368454762,-2.55612121614255));
#58075=CARTESIAN_POINT('Ctrl Pts',(16.1755170133934,-19.040118143674,-2.56242375739948));
#58076=CARTESIAN_POINT('Ctrl Pts',(16.1745315620426,-19.0115058691761,-2.56385246834249));
#58077=CARTESIAN_POINT('Ctrl Pts',(16.1740255308992,-18.9828608310217,-2.5652811792855));
#58078=CARTESIAN_POINT('Ctrl Pts',(16.1740009418753,-18.9541959965583,-2.56670989022851));
#58079=CARTESIAN_POINT('Origin',(18.734,-18.952,1.76670989022851));
#58080=CARTESIAN_POINT('',(20.293535888361,-16.9218650751948,-1.25003886335143));
#58081=CARTESIAN_POINT('',(20.2916962531304,-16.9242237737286,-1.31677679843946));
#58082=CARTESIAN_POINT('',(20.293535888361,-16.9218650751948,1.76670989022851));
#58083=CARTESIAN_POINT('',(16.1742339454204,-18.95300766776,-1.83329006740176));
#58084=CARTESIAN_POINT('Ctrl Pts',(20.2916962531305,-16.9242237737287,-1.31677679843947));
#58085=CARTESIAN_POINT('Ctrl Pts',(20.7197402889178,-17.2576788600888,-1.34369097149553));
#58086=CARTESIAN_POINT('Ctrl Pts',(21.5659317262182,-18.4571855196717,-1.41299708011206));
#58087=CARTESIAN_POINT('Ctrl Pts',(21.0139855935949,-20.9432205334647,-1.52469512428908));
#58088=CARTESIAN_POINT('Ctrl Pts',(18.2938122981759,-21.946916179492,-1.65187093097051));
#58089=CARTESIAN_POINT('Ctrl Pts',(16.4202753042621,-20.536339124494,-1.75473569408312));
#58090=CARTESIAN_POINT('Ctrl Pts',(16.1765569610219,-19.3178333678849,-1.81520852163526));
#58091=CARTESIAN_POINT('Ctrl Pts',(16.1778407221624,-18.9530194401788,-1.83328941362691));
#58092=CARTESIAN_POINT('Ctrl Pts',(16.174000198019,-18.953006904815,-1.8332901097715));
#58093=CARTESIAN_POINT('Ctrl Pts',(16.1739663681252,-18.8669962708809,-1.83754657623655));
#58094=CARTESIAN_POINT('Ctrl Pts',(16.1782715498346,-18.7810104795588,-1.8418030427016));
#58095=CARTESIAN_POINT('Ctrl Pts',(16.186881959491,-18.6955049947587,-1.84605950916664));
#58096=CARTESIAN_POINT('Ctrl Pts',(16.1954973714571,-18.6099498346313,-1.85031844847147));
#58097=CARTESIAN_POINT('Ctrl Pts',(16.2084229438518,-18.5248759665389,-1.85457738777631));
#58098=CARTESIAN_POINT('Ctrl Pts',(16.2255732751413,-18.4407316105854,-1.85883632708114));
#58099=CARTESIAN_POINT('Ctrl Pts',(16.242752034236,-18.3564477798121,-1.86310232585877));
#58100=CARTESIAN_POINT('Ctrl Pts',(16.2641694501873,-18.273096962922,-1.86736832463641));
#58101=CARTESIAN_POINT('Ctrl Pts',(16.2896893999554,-18.1911151923519,-1.87163432341404));
#58102=CARTESIAN_POINT('Ctrl Pts',(16.315231796287,-18.1090613131363,-1.87590407443307));
#58103=CARTESIAN_POINT('Ctrl Pts',(16.3448837660304,-18.02837928517,-1.88017382545211));
#58104=CARTESIAN_POINT('Ctrl Pts',(16.3784607475836,-17.9494857455749,-1.88444357647114));
#58105=CARTESIAN_POINT('Ctrl Pts',(16.4121081360754,-17.8704267756062,-1.88872228065047));
#58106=CARTESIAN_POINT('Ctrl Pts',(16.4496967908486,-17.7931641763823,-1.89300098482979));
#58107=CARTESIAN_POINT('Ctrl Pts',(16.4909957508862,-17.7180907900264,-1.89727968900912));
#58108=CARTESIAN_POINT('Ctrl Pts',(16.5197685295266,-17.6657875377064,-1.90026064078387));
#58109=CARTESIAN_POINT('Ctrl Pts',(16.550341278611,-17.6145463427439,-1.90324159255863));
#58110=CARTESIAN_POINT('Ctrl Pts',(16.582623920045,-17.5644910945881,-1.90622254433338));
#58111=CARTESIAN_POINT('Ctrl Pts',(16.6279420233621,-17.494223953898,-1.91040717962067));
#58112=CARTESIAN_POINT('Ctrl Pts',(16.6767906254559,-17.4260486191802,-1.91459181490796));
#58113=CARTESIAN_POINT('Ctrl Pts',(16.7289503547201,-17.3603417703656,-1.91877645019526));
#58114=CARTESIAN_POINT('Ctrl Pts',(16.7810358412116,-17.2947284469337,-1.92295512918387));
#58115=CARTESIAN_POINT('Ctrl Pts',(16.836422809856,-17.2315769875611,-1.92713380817248));
#58116=CARTESIAN_POINT('Ctrl Pts',(16.8948480567244,-17.1712360825911,-1.93131248716108));
#58117=CARTESIAN_POINT('Ctrl Pts',(16.9543205181339,-17.1098136268105,-1.93556606482166));
#58118=CARTESIAN_POINT('Ctrl Pts',(17.016940988381,-17.0513038784721,-1.93981964248223));
#58119=CARTESIAN_POINT('Ctrl Pts',(17.0823881640359,-16.9960403012068,-1.9440732201428));
#58120=CARTESIAN_POINT('Ctrl Pts',(17.146566536085,-16.94184810136,-1.94824433504437));
#58121=CARTESIAN_POINT('Ctrl Pts',(17.2134626230336,-16.8907776412551,-1.95241544994594));
#58122=CARTESIAN_POINT('Ctrl Pts',(17.282736811581,-16.8431057025209,-1.9565865648475));
#58123=CARTESIAN_POINT('Ctrl Pts',(17.3519877545945,-16.7954497605048,-1.96075628009654));
#58124=CARTESIAN_POINT('Ctrl Pts',(17.4236148357286,-16.7511903355776,-1.96492599534558));
#58125=CARTESIAN_POINT('Ctrl Pts',(17.4972477392747,-16.7105621031153,-1.96909571059463));
#58126=CARTESIAN_POINT('Ctrl Pts',(17.5708780227141,-16.6699353163424,-1.97326527747116));
#58127=CARTESIAN_POINT('Ctrl Pts',(17.6465135834571,-16.6329396866301,-1.97743484434769));
#58128=CARTESIAN_POINT('Ctrl Pts',(17.7237588789704,-16.5997642810762,-1.98160441122423));
#58129=CARTESIAN_POINT('Ctrl Pts',(17.8037199857111,-16.5654224855399,-1.98592057287344));
#58130=CARTESIAN_POINT('Ctrl Pts',(17.8854056436375,-16.5351747548242,-1.99023673452266));
#58131=CARTESIAN_POINT('Ctrl Pts',(17.9683557183502,-16.5091760534216,-1.99455289617187));
#58132=CARTESIAN_POINT('Ctrl Pts',(18.0486037412859,-16.4840242450154,-1.99872846129608));
#58133=CARTESIAN_POINT('Ctrl Pts',(18.1300346026624,-16.4628489694374,-2.00290402642029));
#58134=CARTESIAN_POINT('Ctrl Pts',(18.212219147317,-16.4457388919401,-2.0070795915445));
#58135=CARTESIAN_POINT('Ctrl Pts',(18.2985545773167,-16.4277646377265,-2.01146605145622));
#58136=CARTESIAN_POINT('Ctrl Pts',(18.3857212504153,-16.414277123386,-2.01585251136794));
#58137=CARTESIAN_POINT('Ctrl Pts',(18.4732153214912,-16.4053175793878,-2.02023897127966));
#58138=CARTESIAN_POINT('Ctrl Pts',(18.5607093925672,-16.3963580353896,-2.02462543119138));
#58139=CARTESIAN_POINT('Ctrl Pts',(18.6485302783096,-16.3919264150074,-2.0290118911031));
#58140=CARTESIAN_POINT('Ctrl Pts',(18.7361763184416,-16.3920009250709,-2.03339835101482));
#58141=CARTESIAN_POINT('Ctrl Pts',(18.8197745701694,-16.3920719940094,-2.03758222948031));
#58142=CARTESIAN_POINT('Ctrl Pts',(18.9035248815704,-16.3962424237147,-2.0417661079458));
#58143=CARTESIAN_POINT('Ctrl Pts',(18.9869920193069,-16.4045316413806,-2.04594998641129));
#58144=CARTESIAN_POINT('Ctrl Pts',(19.0703479391413,-16.4128098138685,-2.05012828996194));
#58145=CARTESIAN_POINT('Ctrl Pts',(19.1534209809421,-16.4251958328744,-2.05430659351258));
#58146=CARTESIAN_POINT('Ctrl Pts',(19.2357756009627,-16.4416571456714,-2.05848489706323));
#58147=CARTESIAN_POINT('Ctrl Pts',(19.318045201778,-16.4581014645496,-2.06265888712123));
#58148=CARTESIAN_POINT('Ctrl Pts',(19.3995974052575,-16.4786126315121,-2.06683287717923));
#58149=CARTESIAN_POINT('Ctrl Pts',(19.4800028447553,-16.5031064221537,-2.07100686723723));
#58150=CARTESIAN_POINT('Ctrl Pts',(19.5603542147999,-16.5275837416973,-2.07517805045328));
#58151=CARTESIAN_POINT('Ctrl Pts',(19.6395599135003,-16.5560382324505,-2.07934923366934));
#58152=CARTESIAN_POINT('Ctrl Pts',(19.7172030732731,-16.5883351090507,-2.08352041688539));
#58153=CARTESIAN_POINT('Ctrl Pts',(19.7948145897911,-16.6206188231483,-2.08768990014728));
#58154=CARTESIAN_POINT('Ctrl Pts',(19.8708644093497,-16.6567416327097,-2.09185938340917));
#58155=CARTESIAN_POINT('Ctrl Pts',(19.9449544117899,-16.6965201369627,-2.09602886667105));
#58156=CARTESIAN_POINT('Ctrl Pts',(20.0190582144982,-16.7363060505018,-2.10019912655576));
#58157=CARTESIAN_POINT('Ctrl Pts',(20.0912010629145,-16.7797488058117,-2.10436938644047));
#58158=CARTESIAN_POINT('Ctrl Pts',(20.1610091624569,-16.8266188929361,-2.10853964632518));
#58159=CARTESIAN_POINT('Ctrl Pts',(20.2061939577773,-16.8569565658888,-2.11123893681666));
#58160=CARTESIAN_POINT('Ctrl Pts',(20.2504011024562,-16.8887292250434,-2.11393822730815));
#58161=CARTESIAN_POINT('Ctrl Pts',(20.293535888361,-16.9218650751948,-2.11663751779963));
#58162=CARTESIAN_POINT('',(16.1740004726294,-18.9504444093098,-1.76670989019937));
#58163=CARTESIAN_POINT('Ctrl Pts',(16.1740004726298,-18.9504444087268,-1.7667098902285));
#58164=CARTESIAN_POINT('Ctrl Pts',(16.1740562220874,-18.8586988534878,-1.77129369133236));
#58165=CARTESIAN_POINT('Ctrl Pts',(16.1790436176654,-18.7671041921699,-1.77587749243622));
#58166=CARTESIAN_POINT('Ctrl Pts',(16.1889163327552,-18.6760486877659,-1.78046129354008));
#58167=CARTESIAN_POINT('Ctrl Pts',(16.1979293239818,-18.5929223689306,-1.78464593360694));
#58168=CARTESIAN_POINT('Ctrl Pts',(16.2110359189735,-18.510083390536,-1.78883057367379));
#58169=CARTESIAN_POINT('Ctrl Pts',(16.2282088655394,-18.4279668040492,-1.79301521374065));
#58170=CARTESIAN_POINT('Ctrl Pts',(16.24535736882,-18.3459670990266,-1.79719389755824));
#58171=CARTESIAN_POINT('Ctrl Pts',(16.2665606337553,-18.2646881899744,-1.80137258137583));
#58172=CARTESIAN_POINT('Ctrl Pts',(16.2917396797569,-18.184559755964,-1.80555126519342));
#58173=CARTESIAN_POINT('Ctrl Pts',(16.3173699983022,-18.1029952166205,-1.80980484165292));
#58174=CARTESIAN_POINT('Ctrl Pts',(16.3471199655449,-18.0226232777798,-1.81405841811242));
#58175=CARTESIAN_POINT('Ctrl Pts',(16.3808518405096,-17.9438860483621,-1.81831199457193));
#58176=CARTESIAN_POINT('Ctrl Pts',(16.4139298146452,-17.8666751598207,-1.82248311438838));
#58177=CARTESIAN_POINT('Ctrl Pts',(16.4508365039862,-17.7910366100589,-1.82665423420484));
#58178=CARTESIAN_POINT('Ctrl Pts',(16.4913923920135,-17.7173700487186,-1.8308253540213));
#58179=CARTESIAN_POINT('Ctrl Pts',(16.531934671396,-17.6437282064046,-1.83499507420651));
#58180=CARTESIAN_POINT('Ctrl Pts',(16.5761234959118,-17.5720574410135,-1.83916479439172));
#58181=CARTESIAN_POINT('Ctrl Pts',(16.6237330298035,-17.5027335253662,-1.84333451457693));
#58182=CARTESIAN_POINT('Ctrl Pts',(16.6713408697582,-17.4334120762489,-1.8475040864044));
#58183=CARTESIAN_POINT('Ctrl Pts',(16.7223689159663,-17.3664376895872,-1.85167365823187));
#58184=CARTESIAN_POINT('Ctrl Pts',(16.7765483383152,-17.3021566764789,-1.85584323005933));
#58185=CARTESIAN_POINT('Ctrl Pts',(16.8326324736236,-17.2356158223938,-1.86015938590618));
#58186=CARTESIAN_POINT('Ctrl Pts',(16.8920933527671,-17.1719616497153,-1.86447554175303));
#58187=CARTESIAN_POINT('Ctrl Pts',(16.9545891225287,-17.1115389357183,-1.86879169759988));
#58188=CARTESIAN_POINT('Ctrl Pts',(17.0150492806953,-17.0530843097644,-1.87296726766114));
#58189=CARTESIAN_POINT('Ctrl Pts',(17.0783492743462,-16.9976541389962,-1.87714283772241));
#58190=CARTESIAN_POINT('Ctrl Pts',(17.1441452217407,-16.9455200514219,-1.88131840778368));
#58191=CARTESIAN_POINT('Ctrl Pts',(17.2132640597166,-16.8907530377263,-1.88570485652332));
#58192=CARTESIAN_POINT('Ctrl Pts',(17.2851371188669,-16.8396241343394,-1.89009130526296));
#58193=CARTESIAN_POINT('Ctrl Pts',(17.3593324936003,-16.792396043982,-1.89447775400259));
#58194=CARTESIAN_POINT('Ctrl Pts',(17.4335278683337,-16.7451679536245,-1.89886420274223));
#58195=CARTESIAN_POINT('Ctrl Pts',(17.5100450162907,-16.7018408959928,-1.90325065148187));
#58196=CARTESIAN_POINT('Ctrl Pts',(17.5884257348914,-16.662620257991,-1.90763710022151));
#58197=CARTESIAN_POINT('Ctrl Pts',(17.6632002791341,-16.6252041002441,-1.91182173531041));
#58198=CARTESIAN_POINT('Ctrl Pts',(17.7399490034736,-16.5913855369184,-1.91600637039932));
#58199=CARTESIAN_POINT('Ctrl Pts',(17.8182913485561,-16.5613771385535,-1.92019100548822));
#58200=CARTESIAN_POINT('Ctrl Pts',(17.8965221835584,-16.5314114532183,-1.92436968429646));
#58201=CARTESIAN_POINT('Ctrl Pts',(17.9763417078037,-16.5052453236658,-1.92854836310471));
#58202=CARTESIAN_POINT('Ctrl Pts',(18.0573458795832,-16.4830449171111,-1.93272704191295));
#58203=CARTESIAN_POINT('Ctrl Pts',(18.1398019751916,-16.4604465890842,-1.93698061962086));
#58204=CARTESIAN_POINT('Ctrl Pts',(18.2234851739771,-16.4419577675957,-1.94123419732878));
#58205=CARTESIAN_POINT('Ctrl Pts',(18.3079491747708,-16.427701940277,-1.9454877750367));
#58206=CARTESIAN_POINT('Ctrl Pts',(18.3907756952208,-16.4137224867601,-1.94965888980394));
#58207=CARTESIAN_POINT('Ctrl Pts',(18.4743525389444,-16.403813444343,-1.95383000457117));
#58208=CARTESIAN_POINT('Ctrl Pts',(18.5582464958779,-16.3980401910389,-1.95800111933841));
#58209=CARTESIAN_POINT('Ctrl Pts',(18.642112301844,-16.392268874974,-1.96217083447068));
#58210=CARTESIAN_POINT('Ctrl Pts',(18.7262945511254,-16.390630623423,-1.96634054960296));
#58211=CARTESIAN_POINT('Ctrl Pts',(18.8103550385198,-16.3931389431834,-1.97051026473523));
#58212=CARTESIAN_POINT('Ctrl Pts',(18.8944125351178,-16.3956471737001,-1.9746798315128));
#58213=CARTESIAN_POINT('Ctrl Pts',(18.9783478186395,-16.4023016676252,-1.97884939829037));
#58214=CARTESIAN_POINT('Ctrl Pts',(19.0617241844761,-16.4130638332346,-1.98301896506793));
#58215=CARTESIAN_POINT('Ctrl Pts',(19.1480319248427,-16.4242043787102,-1.98733512688752));
#58216=CARTESIAN_POINT('Ctrl Pts',(19.233740190573,-16.4397467505395,-1.9916512887071));
#58217=CARTESIAN_POINT('Ctrl Pts',(19.3183740371494,-16.4595901250585,-1.99596745052669));
#58218=CARTESIAN_POINT('Ctrl Pts',(19.4002509797579,-16.4787871118714,-2.00014301559772));
#58219=CARTESIAN_POINT('Ctrl Pts',(19.4811219861015,-16.5020090222104,-2.00431858066875));
#58220=CARTESIAN_POINT('Ctrl Pts',(19.560572524251,-16.529113733137,-2.00849414573978));
#58221=CARTESIAN_POINT('Ctrl Pts',(19.6440358680249,-16.5575874207752,-2.01288060593364));
#58222=CARTESIAN_POINT('Ctrl Pts',(19.7259309366168,-16.5903462355689,-2.0172670661275));
#58223=CARTESIAN_POINT('Ctrl Pts',(19.8058030522791,-16.6271692067754,-2.02165352632137));
#58224=CARTESIAN_POINT('Ctrl Pts',(19.8856751679414,-16.6639921779819,-2.02603998651523));
#58225=CARTESIAN_POINT('Ctrl Pts',(19.9635238523658,-16.7048789684718,-2.03042644670909));
#58226=CARTESIAN_POINT('Ctrl Pts',(20.0389283878907,-16.7495554711919,-2.03481290690295));
#58227=CARTESIAN_POINT('Ctrl Pts',(20.1108650768449,-16.7921773063025,-2.03899763425893));
#58228=CARTESIAN_POINT('Ctrl Pts',(20.1808452608001,-16.8384065838528,-2.0431823616149));
#58229=CARTESIAN_POINT('Ctrl Pts',(20.2484841862399,-16.8880383604269,-2.04736708897087));
#58230=CARTESIAN_POINT('Ctrl Pts',(20.2636199533809,-16.8991446133446,-2.04830351808172));
#58231=CARTESIAN_POINT('Ctrl Pts',(20.2786385711608,-16.9104210571001,-2.04923994719258));
#58232=CARTESIAN_POINT('Ctrl Pts',(20.293535888361,-16.9218650751948,-2.05017637630343));
#58233=CARTESIAN_POINT('Ctrl Pts',(20.293535888361,-16.9218650751948,-1.25003886335143));
#58234=CARTESIAN_POINT('Ctrl Pts',(20.360183483879,-16.9730633063139,-1.25422273048467));
#58235=CARTESIAN_POINT('Ctrl Pts',(20.4242257550283,-17.027484305077,-1.25840659761791));
#58236=CARTESIAN_POINT('Ctrl Pts',(20.4853525107207,-17.0848191348474,-1.26259046475115));
#58237=CARTESIAN_POINT('Ctrl Pts',(20.5299990664673,-17.1266960943648,-1.26564633210555));
#58238=CARTESIAN_POINT('Ctrl Pts',(20.5730910166659,-17.1701266981197,-1.26870219945995));
#58239=CARTESIAN_POINT('Ctrl Pts',(20.614521157858,-17.2149795122542,-1.27175806681434));
#58240=CARTESIAN_POINT('Ctrl Pts',(20.6712532028065,-17.2763983680518,-1.2759425952547));
#58241=CARTESIAN_POINT('Ctrl Pts',(20.7250787526129,-17.3407138524111,-1.28012712369507));
#58242=CARTESIAN_POINT('Ctrl Pts',(20.7756877943714,-17.4076195577789,-1.28431165213543));
#58243=CARTESIAN_POINT('Ctrl Pts',(20.8262247790097,-17.4744300028477,-1.28849022264697));
#58244=CARTESIAN_POINT('Ctrl Pts',(20.873554077068,-17.5438229797258,-1.29266879315851));
#58245=CARTESIAN_POINT('Ctrl Pts',(20.9174037166617,-17.6154566187108,-1.29684736367005));
#58246=CARTESIAN_POINT('Ctrl Pts',(20.9620407587122,-17.6883765739313,-1.30110096824612));
#58247=CARTESIAN_POINT('Ctrl Pts',(21.0030716111863,-17.7636181037576,-1.30535457282219));
#58248=CARTESIAN_POINT('Ctrl Pts',(21.04025352208,-17.8407868377789,-1.30960817739827));
#58249=CARTESIAN_POINT('Ctrl Pts',(21.0767133920067,-17.9164570208649,-1.3137791806048));
#58250=CARTESIAN_POINT('Ctrl Pts',(21.1094722614084,-17.9939797943655,-1.31795018381133));
#58251=CARTESIAN_POINT('Ctrl Pts',(21.1383468600458,-18.0729572384759,-1.32212118701787));
#58252=CARTESIAN_POINT('Ctrl Pts',(21.1672117626761,-18.151908162188,-1.32629078961353));
#58253=CARTESIAN_POINT('Ctrl Pts',(21.1921948271095,-18.2323123546668,-1.33046039220919));
#58254=CARTESIAN_POINT('Ctrl Pts',(21.2131612187129,-18.3137526720542,-1.33462999480485));
#58255=CARTESIAN_POINT('Ctrl Pts',(21.2341268601602,-18.3951900755902,-1.33879944821639));
#58256=CARTESIAN_POINT('Ctrl Pts',(21.2510760006384,-18.4776630845829,-1.34296890162792));
#58257=CARTESIAN_POINT('Ctrl Pts',(21.263924266104,-18.560741507724,-1.34713835503945));
#58258=CARTESIAN_POINT('Ctrl Pts',(21.2772250217302,-18.6467457864309,-1.35145464824415));
#58259=CARTESIAN_POINT('Ctrl Pts',(21.2861305792208,-18.7333983970715,-1.35577094144884));
#58260=CARTESIAN_POINT('Ctrl Pts',(21.2906057031231,-18.8202150283278,-1.36008723465354));
#58261=CARTESIAN_POINT('Ctrl Pts',(21.2949348018955,-18.9041987972701,-1.36426268543923));
#58262=CARTESIAN_POINT('Ctrl Pts',(21.2951181997827,-18.9883355761622,-1.36843813622492));
#58263=CARTESIAN_POINT('Ctrl Pts',(21.2911771392428,-19.0721876804588,-1.37261358701061));
#58264=CARTESIAN_POINT('Ctrl Pts',(21.2870366744248,-19.1602824164425,-1.37700030142481));
#58265=CARTESIAN_POINT('Ctrl Pts',(21.2783434340466,-19.2480623296263,-1.381387015839));
#58266=CARTESIAN_POINT('Ctrl Pts',(21.2651832590201,-19.3350291232487,-1.3857737302532));
#58267=CARTESIAN_POINT('Ctrl Pts',(21.2520230839935,-19.421995916871,-1.39016044466739));
#58268=CARTESIAN_POINT('Ctrl Pts',(21.2343961652463,-19.5081490374756,-1.39454715908158));
#58269=CARTESIAN_POINT('Ctrl Pts',(21.2124488480671,-19.5930080401328,-1.39893387349578));
#58270=CARTESIAN_POINT('Ctrl Pts',(21.1915123903351,-19.6739585685189,-1.40311854263622));
#58271=CARTESIAN_POINT('Ctrl Pts',(21.166566824132,-19.7540329106642,-1.40730321177665));
#58272=CARTESIAN_POINT('Ctrl Pts',(21.1377020187579,-19.8328045214571,-1.41148788091709));
#58273=CARTESIAN_POINT('Ctrl Pts',(21.1088782963373,-19.9114640175003,-1.41566659406489));
#58274=CARTESIAN_POINT('Ctrl Pts',(21.0761465717546,-19.9888240368999,-1.41984530721269));
#58275=CARTESIAN_POINT('Ctrl Pts',(21.0396471223768,-20.0644708297639,-1.42402402036049));
#58276=CARTESIAN_POINT('Ctrl Pts',(21.0024938345812,-20.1414727329157,-1.42827758951952));
#58277=CARTESIAN_POINT('Ctrl Pts',(20.9614366228418,-20.2166989566014,-1.43253115867855));
#58278=CARTESIAN_POINT('Ctrl Pts',(20.9166756992289,-20.2897319582023,-1.43678472783758));
#58279=CARTESIAN_POINT('Ctrl Pts',(20.8727820889758,-20.361349830425,-1.44095587739797));
#58280=CARTESIAN_POINT('Ctrl Pts',(20.8253272686825,-20.4308583065096,-1.44512702695836));
#58281=CARTESIAN_POINT('Ctrl Pts',(20.7745466530899,-20.4978878861559,-1.44929817651875));
#58282=CARTESIAN_POINT('Ctrl Pts',(20.723783075874,-20.5648949754245,-1.45346792653688));
#58283=CARTESIAN_POINT('Ctrl Pts',(20.6696961971179,-20.6294244537336,-1.45763767655502));
#58284=CARTESIAN_POINT('Ctrl Pts',(20.6125638119978,-20.6911371436009,-1.46180742657315));
#58285=CARTESIAN_POINT('Ctrl Pts',(20.5554334589444,-20.7528476384907,-1.46597702828293));
#58286=CARTESIAN_POINT('Ctrl Pts',(20.4952581280413,-20.8117412071425,-1.47014662999271));
#58287=CARTESIAN_POINT('Ctrl Pts',(20.4323538975484,-20.867514040325,-1.47431623170249));
#58288=CARTESIAN_POINT('Ctrl Pts',(20.3672392245803,-20.9252467200626,-1.47863235240872));
#58289=CARTESIAN_POINT('Ctrl Pts',(20.299200687246,-20.9796349039107,-1.48294847311494));
#58290=CARTESIAN_POINT('Ctrl Pts',(20.2286263802879,-21.0303868704713,-1.48726459382117));
#58291=CARTESIAN_POINT('Ctrl Pts',(20.1603497774659,-21.0794864934453,-1.4914401935811));
#58292=CARTESIAN_POINT('Ctrl Pts',(20.089700407782,-21.1251828200969,-1.49561579334102));
#58293=CARTESIAN_POINT('Ctrl Pts',(20.0170578148023,-21.1672567896013,-1.49979139310095));
#58294=CARTESIAN_POINT('Ctrl Pts',(19.940748273422,-21.2114546243045,-1.50417777428033));
#58295=CARTESIAN_POINT('Ctrl Pts',(19.8622394999333,-21.251654504136,-1.5085641554597));
#58296=CARTESIAN_POINT('Ctrl Pts',(19.7819968158146,-21.287658937868,-1.51295053663908));
#58297=CARTESIAN_POINT('Ctrl Pts',(19.7017541316958,-21.3236633715999,-1.51733691781846));
#58298=CARTESIAN_POINT('Ctrl Pts',(19.6197781052968,-21.3554722202674,-1.52172329899784));
#58299=CARTESIAN_POINT('Ctrl Pts',(19.5365517913642,-21.3829485025763,-1.52610968017722));
#58300=CARTESIAN_POINT('Ctrl Pts',(19.4571532093435,-21.4091610999082,-1.53029432358371));
#58301=CARTESIAN_POINT('Ctrl Pts',(19.376321311697,-21.4315284613918,-1.53447896699021));
#58302=CARTESIAN_POINT('Ctrl Pts',(19.294463394386,-21.4498952707336,-1.53866361039671));
#58303=CARTESIAN_POINT('Ctrl Pts',(19.2127219863795,-21.4682359383869,-1.54284229775267));
#58304=CARTESIAN_POINT('Ctrl Pts',(19.1299579044461,-21.4825872641847,-1.54702098510862));
#58305=CARTESIAN_POINT('Ctrl Pts',(19.0465949711256,-21.4928432427104,-1.55119967246457));
#58306=CARTESIAN_POINT('Ctrl Pts',(18.9617380510235,-21.5032830235057,-1.55545324806433));
#58307=CARTESIAN_POINT('Ctrl Pts',(18.8762610608014,-21.5094790670078,-1.55970682366408));
#58308=CARTESIAN_POINT('Ctrl Pts',(18.7906234643,-21.5113737091896,-1.56396039926383));
#58309=CARTESIAN_POINT('Ctrl Pts',(18.7066458764304,-21.5132316254179,-1.56813152308422));
#58310=CARTESIAN_POINT('Ctrl Pts',(18.6225143342412,-21.5109533994767,-1.5723026469046));
#58311=CARTESIAN_POINT('Ctrl Pts',(18.5386669500421,-21.5045369732081,-1.57647377072499));
#58312=CARTESIAN_POINT('Ctrl Pts',(18.4548476977165,-21.4981226997328,-1.5806434950798));
#58313=CARTESIAN_POINT('Ctrl Pts',(18.3713128723448,-21.4875730184253,-1.58481321943461));
#58314=CARTESIAN_POINT('Ctrl Pts',(18.2884980293892,-21.4729379195414,-1.58898294378941));
#58315=CARTESIAN_POINT('Ctrl Pts',(18.2056861297709,-21.4583033408063,-1.59315251994729));
#58316=CARTESIAN_POINT('Ctrl Pts',(18.1235946145539,-21.4395837140867,-1.59732209610518));
#58317=CARTESIAN_POINT('Ctrl Pts',(18.0426500220353,-21.4168803638246,-1.60149167226306));
#58318=CARTESIAN_POINT('Ctrl Pts',(17.9588599464441,-21.3933789120853,-1.60580782347935));
#58319=CARTESIAN_POINT('Ctrl Pts',(17.8762994409707,-21.3656085753716,-1.61012397469565));
#58320=CARTESIAN_POINT('Ctrl Pts',(17.7954238784078,-21.3337377823717,-1.61444012591195));
#58321=CARTESIAN_POINT('Ctrl Pts',(17.7171824220401,-21.3029050168134,-1.61861570066365));
#58322=CARTESIAN_POINT('Ctrl Pts',(17.6405182464777,-21.2682350343783,-1.62279127541534));
#58323=CARTESIAN_POINT('Ctrl Pts',(17.5658209821028,-21.2299283970627,-1.62696685016703));
#58324=CARTESIAN_POINT('Ctrl Pts',(17.4873515385791,-21.1896872913332,-1.63135328961563));
#58325=CARTESIAN_POINT('Ctrl Pts',(17.4110533971718,-21.1454328556654,-1.63573972906424));
#58326=CARTESIAN_POINT('Ctrl Pts',(17.3373445042313,-21.097449469491,-1.64012616851284));
#58327=CARTESIAN_POINT('Ctrl Pts',(17.2636356112909,-21.0494660833166,-1.64451260796144));
#58328=CARTESIAN_POINT('Ctrl Pts',(17.1925163913427,-20.9977541493591,-1.64889904741004));
#58329=CARTESIAN_POINT('Ctrl Pts',(17.1243635064003,-20.9426457139511,-1.65328548685865));
#58330=CARTESIAN_POINT('Ctrl Pts',(17.0601943718463,-20.8907585398463,-1.6574155251311));
#58331=CARTESIAN_POINT('Ctrl Pts',(16.9984022164044,-20.8356563912925,-1.66154556340355));
#58332=CARTESIAN_POINT('Ctrl Pts',(16.9393333497915,-20.7775880188667,-1.66567560167601));
#58333=CARTESIAN_POINT('Ctrl Pts',(16.8791242536685,-20.7183987298625,-1.66988536369781));
#58334=CARTESIAN_POINT('Ctrl Pts',(16.8217451259872,-20.6561277338344,-1.67409512571962));
#58335=CARTESIAN_POINT('Ctrl Pts',(16.7675298313412,-20.5910836085371,-1.67830488774143));
#58336=CARTESIAN_POINT('Ctrl Pts',(16.7144792342514,-20.5274368146437,-1.6824242121926));
#58337=CARTESIAN_POINT('Ctrl Pts',(16.6644582227548,-20.4611352262018,-1.68654353664378));
#58338=CARTESIAN_POINT('Ctrl Pts',(16.6177431437369,-20.3925057855904,-1.69066286109495));
#58339=CARTESIAN_POINT('Ctrl Pts',(16.5710563620564,-20.3239179167901,-1.69477969029369));
#58340=CARTESIAN_POINT('Ctrl Pts',(16.5276718049372,-20.2530053838409,-1.69889651949243));
#58341=CARTESIAN_POINT('Ctrl Pts',(16.4878244177667,-20.1801267254559,-1.70301334869118));
#58342=CARTESIAN_POINT('Ctrl Pts',(16.4479884749074,-20.1072689980804,-1.70712899552195));
#58343=CARTESIAN_POINT('Ctrl Pts',(16.4116879114515,-20.0324466815215,-1.71124464235271));
#58344=CARTESIAN_POINT('Ctrl Pts',(16.3791125478311,-19.9560443653632,-1.71536028918348));
#58345=CARTESIAN_POINT('Ctrl Pts',(16.3452431871199,-19.8766071061112,-1.71963942260147));
#58346=CARTESIAN_POINT('Ctrl Pts',(16.3154014154543,-19.795462185038,-1.72391855601946));
#58347=CARTESIAN_POINT('Ctrl Pts',(16.28974541526,-19.7130647311349,-1.72819768943746));
#58348=CARTESIAN_POINT('Ctrl Pts',(16.2650470315947,-19.6337427825017,-1.73231710314623));
#58349=CARTESIAN_POINT('Ctrl Pts',(16.2442275676729,-19.5532606331567,-1.736436516855));
#58350=CARTESIAN_POINT('Ctrl Pts',(16.2273766226977,-19.4720377335941,-1.74055593056377));
#58351=CARTESIAN_POINT('Ctrl Pts',(16.2105163820987,-19.3907700283831,-1.74467761669822));
#58352=CARTESIAN_POINT('Ctrl Pts',(16.1976290876222,-19.3087612270287,-1.74879930283266));
#58353=CARTESIAN_POINT('Ctrl Pts',(16.1887526585032,-19.2264375531951,-1.7529209889671));
#58354=CARTESIAN_POINT('Ctrl Pts',(16.1798641546722,-19.1440018934889,-1.75704828188022));
#58355=CARTESIAN_POINT('Ctrl Pts',(16.1749974203025,-19.0612509779236,-1.76117557479333));
#58356=CARTESIAN_POINT('Ctrl Pts',(16.174138321227,-18.9786117558525,-1.76530286770644));
#58357=CARTESIAN_POINT('Ctrl Pts',(16.1740406969692,-18.9692209964452,-1.76577187520409));
#58358=CARTESIAN_POINT('Ctrl Pts',(16.1739947684326,-18.9598316737892,-1.76624088270173));
#58359=CARTESIAN_POINT('Ctrl Pts',(16.1740004726294,-18.9504444093098,-1.76670989019937));
#58360=CARTESIAN_POINT('Origin',(18.734,-18.952,1.76670989022851));
#58361=CARTESIAN_POINT('',(20.2910039261765,-16.9251777670034,-0.450077510764929));
#58362=CARTESIAN_POINT('',(20.2957383198016,-16.919032322281,-0.51674866945634));
#58363=CARTESIAN_POINT('',(20.293535888361,-16.9218650751948,1.76670989022851));
#58364=CARTESIAN_POINT('',(16.1765334791563,-18.9551432954109,-0.166709890228505));
#58365=CARTESIAN_POINT('Ctrl Pts',(16.1765334791563,-18.9551432954109,-0.166709890228505));
#58366=CARTESIAN_POINT('Ctrl Pts',(16.1810511645957,-18.366678437132,-0.195923797939959));
#58367=CARTESIAN_POINT('Ctrl Pts',(16.6739009874383,-16.9152607583549,-0.267529641211892));
#58368=CARTESIAN_POINT('Ctrl Pts',(18.6725570461647,-16.1123849326032,-0.361985514724032));
#58369=CARTESIAN_POINT('Ctrl Pts',(19.9247548372555,-16.6451525276585,-0.42722748052472));
#58370=CARTESIAN_POINT('Ctrl Pts',(20.2910039261765,-16.9251777670034,-0.450077510764929));
#58371=CARTESIAN_POINT('',(18.0722627314315,-21.4249949024184,0.));
#58372=CARTESIAN_POINT('Ctrl Pts',(18.0722627314315,-21.4249949024184,8.32667268468867E-16));
#58373=CARTESIAN_POINT('Ctrl Pts',(17.2488902483963,-21.2046724677036,-0.0423919355604773));
#58374=CARTESIAN_POINT('Ctrl Pts',(16.3345567445347,-20.3367913268265,-0.0979618989699792));
#58375=CARTESIAN_POINT('Ctrl Pts',(16.174495607841,-19.2205924221476,-0.153531862379481));
#58376=CARTESIAN_POINT('Ctrl Pts',(16.1765334791563,-18.9551432954109,-0.166709890228505));
#58377=CARTESIAN_POINT('',(19.3957675194894,-21.4249868075161,-1.730088294849E-11));
#58378=CARTESIAN_POINT('Origin',(18.734,-18.952,0.));
#58379=CARTESIAN_POINT('',(16.1740007446509,-18.9500474088581,-0.233290109771496));
#58380=CARTESIAN_POINT('Ctrl Pts',(19.3957675194894,-21.4249868075161,-1.73008274373387E-11));
#58381=CARTESIAN_POINT('Ctrl Pts',(19.3150528143647,-21.4465859402064,-0.00418159702990585));
#58382=CARTESIAN_POINT('Ctrl Pts',(19.2331283755591,-21.4642697491679,-0.0083631940425111));
#58383=CARTESIAN_POINT('Ctrl Pts',(19.1504091626665,-21.4779064529882,-0.0125447910551162));
#58384=CARTESIAN_POINT('Ctrl Pts',(19.0678077425558,-21.4915237380395,-0.0167204334420983));
#58385=CARTESIAN_POINT('Ctrl Pts',(18.9844142470727,-21.501105290632,-0.0208960758290806));
#58386=CARTESIAN_POINT('Ctrl Pts',(18.9006573352602,-21.506569500445,-0.0250717182160627));
#58387=CARTESIAN_POINT('Ctrl Pts',(18.8165041727153,-21.5120595612247,-0.029267115406781));
#58388=CARTESIAN_POINT('Ctrl Pts',(18.7319846004062,-21.5133930928997,-0.0334625125974991));
#58389=CARTESIAN_POINT('Ctrl Pts',(18.6475423362417,-21.5105396366634,-0.0376579097882175));
#58390=CARTESIAN_POINT('Ctrl Pts',(18.5636493303861,-21.5077047408548,-0.041826017838971));
#58391=CARTESIAN_POINT('Ctrl Pts',(18.4798330960835,-21.5007371781061,-0.0459941258897243));
#58392=CARTESIAN_POINT('Ctrl Pts',(18.3965306502634,-21.4896592438679,-0.0501622339404779));
#58393=CARTESIAN_POINT('Ctrl Pts',(18.3132562868314,-21.4785850441522,-0.0543289368652889));
#58394=CARTESIAN_POINT('Ctrl Pts',(18.2304958242585,-21.4634032856077,-0.0584956397901002));
#58395=CARTESIAN_POINT('Ctrl Pts',(18.1486808249577,-21.4441880874701,-0.0626623427149111));
#58396=CARTESIAN_POINT('Ctrl Pts',(18.0668687681529,-21.4249735804117,-0.0668288957832525));
#58397=CARTESIAN_POINT('Ctrl Pts',(17.9860025553434,-21.4017260285035,-0.0709954488515935));
#58398=CARTESIAN_POINT('Ctrl Pts',(17.9065018743522,-21.3745702986806,-0.0751620019199348));
#58399=CARTESIAN_POINT('Ctrl Pts',(17.8260461859792,-21.3470883587911,-0.0793786059927156));
#58400=CARTESIAN_POINT('Ctrl Pts',(17.7469895187101,-21.3156038569086,-0.0835952100654965));
#58401=CARTESIAN_POINT('Ctrl Pts',(17.6697476372837,-21.2802969974753,-0.0878118141382773));
#58402=CARTESIAN_POINT('Ctrl Pts',(17.5933153937669,-21.24536021929,-0.0919842203944796));
#58403=CARTESIAN_POINT('Ctrl Pts',(17.5186604552654,-21.2066811083584,-0.0961566266506819));
#58404=CARTESIAN_POINT('Ctrl Pts',(17.4461606843492,-21.1644804851262,-0.100329032906884));
#58405=CARTESIAN_POINT('Ctrl Pts',(17.3725089409092,-21.1216093224172,-0.104567735887954));
#58406=CARTESIAN_POINT('Ctrl Pts',(17.3010818658164,-21.0751040329196,-0.108806438869025));
#58407=CARTESIAN_POINT('Ctrl Pts',(17.2322432557832,-21.0252406230824,-0.113045141850095));
#58408=CARTESIAN_POINT('Ctrl Pts',(17.1634046457499,-20.9753772132452,-0.117283844831166));
#58409=CARTESIAN_POINT('Ctrl Pts',(17.0971548434137,-20.922156041386,-0.121522547812235));
#58410=CARTESIAN_POINT('Ctrl Pts',(17.0338195258261,-20.8658929842699,-0.125761250793306));
#58411=CARTESIAN_POINT('Ctrl Pts',(16.9721381141262,-20.8110991516714,-0.129889266466191));
#58412=CARTESIAN_POINT('Ctrl Pts',(16.9129812124539,-20.7532072684117,-0.134017282139077));
#58413=CARTESIAN_POINT('Ctrl Pts',(16.8566825230424,-20.6924824304513,-0.138145297811962));
#58414=CARTESIAN_POINT('Ctrl Pts',(16.8004749041019,-20.6318558228343,-0.142266635881243));
#58415=CARTESIAN_POINT('Ctrl Pts',(16.7471166297386,-20.5684057102785,-0.146387973950524));
#58416=CARTESIAN_POINT('Ctrl Pts',(16.6969071781283,-20.5024363369964,-0.150509312019806));
#58417=CARTESIAN_POINT('Ctrl Pts',(16.6467433529369,-20.4365269115162,-0.154626904939698));
#58418=CARTESIAN_POINT('Ctrl Pts',(16.5997229596986,-20.3681031412178,-0.158744497859592));
#58419=CARTESIAN_POINT('Ctrl Pts',(16.556106820746,-20.2975041061843,-0.162862090779484));
#58420=CARTESIAN_POINT('Ctrl Pts',(16.5125163940206,-20.2269466901128,-0.166977256329893));
#58421=CARTESIAN_POINT('Ctrl Pts',(16.4723264872833,-20.1542169560892,-0.171092421880302));
#58422=CARTESIAN_POINT('Ctrl Pts',(16.4357550860861,-20.0796836061897,-0.175207587430711));
#58423=CARTESIAN_POINT('Ctrl Pts',(16.3991935731796,-20.005170408852,-0.179321640309701));
#58424=CARTESIAN_POINT('Ctrl Pts',(16.3662488306016,-19.9288549893914,-0.18343569318869));
#58425=CARTESIAN_POINT('Ctrl Pts',(16.3370925482441,-19.8511299504059,-0.18754974606768));
#58426=CARTESIAN_POINT('Ctrl Pts',(16.3079200305593,-19.7733616311617,-0.191666089807838));
#58427=CARTESIAN_POINT('Ctrl Pts',(16.2825403576348,-19.694182567114,-0.195782433547997));
#58428=CARTESIAN_POINT('Ctrl Pts',(16.2610764230542,-19.6140037632713,-0.199898777288155));
#58429=CARTESIAN_POINT('Ctrl Pts',(16.239606571648,-19.5338028570508,-0.204016255754456));
#58430=CARTESIAN_POINT('Ctrl Pts',(16.2220547122219,-19.4526021247793,-0.208133734220756));
#58431=CARTESIAN_POINT('Ctrl Pts',(16.2084928022863,-19.3708238225034,-0.212251212687057));
#58432=CARTESIAN_POINT('Ctrl Pts',(16.1949128185011,-19.2889365349339,-0.216374178484198));
#58433=CARTESIAN_POINT('Ctrl Pts',(16.1853334601433,-19.2064706109328,-0.22049714428134));
#58434=CARTESIAN_POINT('Ctrl Pts',(16.1797748249049,-19.1238538766228,-0.224620110078481));
#58435=CARTESIAN_POINT('Ctrl Pts',(16.1758784900672,-19.0659435359969,-0.227510109976153));
#58436=CARTESIAN_POINT('Ctrl Pts',(16.1739565735353,-19.0079591859799,-0.230400109873824));
#58437=CARTESIAN_POINT('Ctrl Pts',(16.1740007446509,-18.9500474088581,-0.233290109771496));
#58438=CARTESIAN_POINT('Ctrl Pts',(16.1719919811635,-18.9500458767116,-0.233290109771496));
#58439=CARTESIAN_POINT('Ctrl Pts',(16.1708576376271,-18.8187090077496,-0.239839092339242));
#58440=CARTESIAN_POINT('Ctrl Pts',(16.2398215302323,-17.838374208454,-0.288780010467466));
#58441=CARTESIAN_POINT('Ctrl Pts',(17.5061738910726,-16.184820909787,-0.380112864156167));
#58442=CARTESIAN_POINT('Ctrl Pts',(19.5043144349347,-16.3488645227434,-0.468050068150036));
#58443=CARTESIAN_POINT('Ctrl Pts',(20.245887371914,-16.8802618854419,-0.513595336583427));
#58444=CARTESIAN_POINT('Ctrl Pts',(20.2957383198016,-16.919032322281,-0.51674866945634));
#58445=CARTESIAN_POINT('Origin',(-18.734,-18.952,1.76670989022851));
#58446=CARTESIAN_POINT('',(-17.1724222329607,-16.9192441176791,-21.2501821957929));
#58447=CARTESIAN_POINT('',(-17.1763092963127,-16.9243021577154,-21.3166133914793));
#58448=CARTESIAN_POINT('',(-17.1744641548914,-16.9218650419685,1.76670989022851));
#58449=CARTESIAN_POINT('',(-21.2914666104891,-18.9488558930302,-21.8332901097715));
#58450=CARTESIAN_POINT('Ctrl Pts',(-17.1763092963129,-16.9243021577153,
-21.3166133914793));
#58451=CARTESIAN_POINT('Ctrl Pts',(-16.9218454642793,-17.1171758532038,
-21.3324492498505));
#58452=CARTESIAN_POINT('Ctrl Pts',(-16.1161224117162,-17.9919927187592,
-21.3906770437821));
#58453=CARTESIAN_POINT('Ctrl Pts',(-16.015951839906,-20.2843427864635,-21.4912967732743));
#58454=CARTESIAN_POINT('Ctrl Pts',(-18.3819425515704,-21.9577205200055,
-21.6184725799557));
#58455=CARTESIAN_POINT('Ctrl Pts',(-20.7940987275605,-20.9887402433146,
-21.7324703587881));
#58456=CARTESIAN_POINT('Ctrl Pts',(-21.2869488458059,-19.5373211115314,
-21.80407620206));
#58457=CARTESIAN_POINT('Ctrl Pts',(-21.2914666104891,-18.9488558930302,
-21.8332901097715));
#58458=CARTESIAN_POINT('',(-19.3957372685685,-16.4790050975816,-22.));
#58459=CARTESIAN_POINT('Ctrl Pts',(-21.2914666104891,-18.9488558930302,
-21.8332901097715));
#58460=CARTESIAN_POINT('Ctrl Pts',(-21.2935045175504,-18.6834066038016,
-21.8464681376205));
#58461=CARTESIAN_POINT('Ctrl Pts',(-21.1334434961762,-17.5672072134799,
-21.90203810103));
#58462=CARTESIAN_POINT('Ctrl Pts',(-20.2191097516036,-16.6993275322964,
-21.9576080644395));
#58463=CARTESIAN_POINT('Ctrl Pts',(-19.3957372685685,-16.4790050975816,
-22.));
#58464=CARTESIAN_POINT('',(-18.072232390111,-16.4790132166747,-21.9999999999826));
#58465=CARTESIAN_POINT('Origin',(-18.734,-18.952,-22.));
#58466=CARTESIAN_POINT('',(-21.2939992553327,-18.9539526125931,-21.7667098902285));
#58467=CARTESIAN_POINT('Ctrl Pts',(-21.2939992553327,-18.9539526125931,
-21.7667098902285));
#58468=CARTESIAN_POINT('Ctrl Pts',(-21.2940622837578,-18.8713183400037,
-21.7708336287807));
#58469=CARTESIAN_POINT('Ctrl Pts',(-21.290120073806,-18.7885361132696,-21.7749573673329));
#58470=CARTESIAN_POINT('Ctrl Pts',(-21.2821561914378,-18.7060324736127,
-21.7790811058851));
#58471=CARTESIAN_POINT('Ctrl Pts',(-21.2742021133718,-18.6236304038401,
-21.7831997677201));
#58472=CARTESIAN_POINT('Ctrl Pts',(-21.2622362429578,-18.5415067083406,
-21.7873184295551));
#58473=CARTESIAN_POINT('Ctrl Pts',(-21.2462941819498,-18.4600874637281,
-21.7914370913901));
#58474=CARTESIAN_POINT('Ctrl Pts',(-21.2303628128015,-18.3787228245485,
-21.7955529909627));
#58475=CARTESIAN_POINT('Ctrl Pts',(-21.2104606337788,-18.2980621623454,
-21.7996688905354));
#58476=CARTESIAN_POINT('Ctrl Pts',(-21.1866748711293,-18.2185247267081,
-21.803784790108));
#58477=CARTESIAN_POINT('Ctrl Pts',(-21.1628974701717,-18.1390152518109,
-21.8078992427696));
#58478=CARTESIAN_POINT('Ctrl Pts',(-21.1352393308965,-18.0606286731435,
-21.8120136954312));
#58479=CARTESIAN_POINT('Ctrl Pts',(-21.1038380346635,-17.9837708486818,
-21.8161281480927));
#58480=CARTESIAN_POINT('Ctrl Pts',(-21.0724377570491,-17.9069155173914,
-21.8202424672866));
#58481=CARTESIAN_POINT('Ctrl Pts',(-21.0372947445442,-17.8315892795539,
-21.8243567864805));
#58482=CARTESIAN_POINT('Ctrl Pts',(-20.9985948099081,-17.758178259983,-21.8284711056744));
#58483=CARTESIAN_POINT('Ctrl Pts',(-20.959859225451,-17.6846996152406,-21.8325892149197));
#58484=CARTESIAN_POINT('Ctrl Pts',(-20.9175603979486,-17.613140131245,-21.836707324165));
#58485=CARTESIAN_POINT('Ctrl Pts',(-20.8719298849008,-17.5438608707773,
-21.8408254334103));
#58486=CARTESIAN_POINT('Ctrl Pts',(-20.8262774812034,-17.4745483744787,
-21.8449455182654));
#58487=CARTESIAN_POINT('Ctrl Pts',(-20.7772904911253,-17.4075186609022,
-21.8490656031205));
#58488=CARTESIAN_POINT('Ctrl Pts',(-20.7252420557879,-17.3431012849587,
-21.8531856879756));
#58489=CARTESIAN_POINT('Ctrl Pts',(-20.6731075913472,-17.2785774357072,
-21.85731258278));
#58490=CARTESIAN_POINT('Ctrl Pts',(-20.6179018945763,-17.2166748979188,
-21.8614394775843));
#58491=CARTESIAN_POINT('Ctrl Pts',(-20.5599360513378,-17.1576874473981,
-21.8655663723887));
#58492=CARTESIAN_POINT('Ctrl Pts',(-20.5193323481527,-17.1163681324571,
-21.8684571646614));
#58493=CARTESIAN_POINT('Ctrl Pts',(-20.4773751065851,-17.076478372295,-21.871347956934));
#58494=CARTESIAN_POINT('Ctrl Pts',(-20.4341804678598,-17.0381070101209,
-21.8742387492067));
#58495=CARTESIAN_POINT('Ctrl Pts',(-20.3717052812394,-16.9826080388726,
-21.8784198881639));
#58496=CARTESIAN_POINT('Ctrl Pts',(-20.3063943198782,-16.9300688092441,
-21.8826010271211));
#58497=CARTESIAN_POINT('Ctrl Pts',(-20.2385599097816,-16.8807927486903,
-21.8867821660783));
#58498=CARTESIAN_POINT('Ctrl Pts',(-20.1708205215985,-16.8315857136584,
-21.8909574481286));
#58499=CARTESIAN_POINT('Ctrl Pts',(-20.1005650755227,-16.7856330369313,
-21.8951327301788));
#58500=CARTESIAN_POINT('Ctrl Pts',(-20.0281405702344,-16.7431993787412,
-21.8993080122291));
#58501=CARTESIAN_POINT('Ctrl Pts',(-19.9553653729372,-16.7005602494225,
-21.9035035117188));
#58502=CARTESIAN_POINT('Ctrl Pts',(-19.880400404287,-16.6614746253178,-21.9076990112086));
#58503=CARTESIAN_POINT('Ctrl Pts',(-19.8036290904368,-16.6261681898961,
-21.9118945106983));
#58504=CARTESIAN_POINT('Ctrl Pts',(-19.7273611982937,-16.5910932735809,
-21.916062498538));
#58505=CARTESIAN_POINT('Ctrl Pts',(-19.6493110036014,-16.5597483260403,
-21.9202304863778));
#58506=CARTESIAN_POINT('Ctrl Pts',(-19.5698794212801,-16.5323087814598,
-21.9243984742175));
#58507=CARTESIAN_POINT('Ctrl Pts',(-19.4904728949047,-16.5048778924257,
-21.9285651473047));
#58508=CARTESIAN_POINT('Ctrl Pts',(-19.4096862815083,-16.4813501100524,
-21.9327318203918));
#58509=CARTESIAN_POINT('Ctrl Pts',(-19.3279387681294,-16.4618520646932,
-21.936898493479));
#58510=CARTESIAN_POINT('Ctrl Pts',(-19.2461924230011,-16.4423542979797,
-21.9410651070204));
#58511=CARTESIAN_POINT('Ctrl Pts',(-19.1634856536714,-16.4268862595724,
-21.9452317205618));
#58512=CARTESIAN_POINT('Ctrl Pts',(-19.0802496942046,-16.415523871734,-21.9493983341032));
#58513=CARTESIAN_POINT('Ctrl Pts',(-18.9960110559548,-16.4040246100579,
-21.9536151395932));
#58514=CARTESIAN_POINT('Ctrl Pts',(-18.9112308686983,-16.39673065975,-21.9578319450831));
#58515=CARTESIAN_POINT('Ctrl Pts',(-18.8263615920593,-16.3936666878,-21.962048750573));
#58516=CARTESIAN_POINT('Ctrl Pts',(-18.742380245673,-16.3906347721311,-21.9662214384587));
#58517=CARTESIAN_POINT('Ctrl Pts',(-18.6583121305892,-16.3917446684187,
-21.9703941263443));
#58518=CARTESIAN_POINT('Ctrl Pts',(-18.5745939384244,-16.3969677678094,
-21.97456681423));
#58519=CARTESIAN_POINT('Ctrl Pts',(-18.4895480243537,-16.402273702523,-21.9788056785221));
#58520=CARTESIAN_POINT('Ctrl Pts',(-18.4048637212048,-16.4118243850528,
-21.9830445428142));
#58521=CARTESIAN_POINT('Ctrl Pts',(-18.3209897195339,-16.4255355715488,
-21.9872834071063));
#58522=CARTESIAN_POINT('Ctrl Pts',(-18.237115717863,-16.4392467580448,-21.9915222713984));
#58523=CARTESIAN_POINT('Ctrl Pts',(-18.1540524839651,-16.4571182804316,
-21.9957611356905));
#58524=CARTESIAN_POINT('Ctrl Pts',(-18.072232390111,-16.4790132166747,-21.9999999999825));
#58525=CARTESIAN_POINT('Ctrl Pts',(-17.1724222329607,-16.9192441176791,
-21.2501821957929));
#58526=CARTESIAN_POINT('Ctrl Pts',(-16.5648621340115,-17.3928060882893,
-21.2886333046889));
#58527=CARTESIAN_POINT('Ctrl Pts',(-15.7493320480079,-19.0034153957527,
-21.3694763491455));
#58528=CARTESIAN_POINT('Ctrl Pts',(-17.0720919824152,-21.4819373889294,
-21.4927113291624));
#58529=CARTESIAN_POINT('Ctrl Pts',(-19.9618261650098,-21.7191790573139,
-21.6198871358439));
#58530=CARTESIAN_POINT('Ctrl Pts',(-21.2281784624135,-20.0656258695291,
-21.7112199895325));
#58531=CARTESIAN_POINT('Ctrl Pts',(-21.297142385429,-19.0852910214283,-21.7601609076607));
#58532=CARTESIAN_POINT('Ctrl Pts',(-21.2960080465361,-18.9539541447775,
-21.7667098902285));
#58533=CARTESIAN_POINT('Origin',(-18.734,-18.952,1.76670989022851));
#58534=CARTESIAN_POINT('',(-17.1739275304994,-16.9211547578705,-20.4499991767297));
#58535=CARTESIAN_POINT('',(-17.1744641548914,-16.9218650419685,-20.5167504990879));
#58536=CARTESIAN_POINT('',(-17.1744641548914,-16.9218650419685,1.76670989022851));
#58537=CARTESIAN_POINT('',(-21.2939288361815,-18.9533417016661,-21.0332900817679));
#58538=CARTESIAN_POINT('Ctrl Pts',(-17.1744641548914,-16.9218650419685,
-20.5167504990879));
#58539=CARTESIAN_POINT('Ctrl Pts',(-17.1078270588004,-16.9730552052415,
-20.5209209383463));
#58540=CARTESIAN_POINT('Ctrl Pts',(-17.0436731835532,-17.0275603476493,
-20.5250913776047));
#58541=CARTESIAN_POINT('Ctrl Pts',(-16.9823431362282,-17.0851046543523,
-20.529261816863));
#58542=CARTESIAN_POINT('Ctrl Pts',(-16.9210263043821,-17.1426365613327,
-20.5334313574697));
#58543=CARTESIAN_POINT('Ctrl Pts',(-16.8625324269728,-17.2032060169337,
-20.5376008980763));
#58544=CARTESIAN_POINT('Ctrl Pts',(-16.8071670928462,-17.2664986063758,
-20.541770438683));
#58545=CARTESIAN_POINT('Ctrl Pts',(-16.7517970815659,-17.3297965426503,
-20.5459403315241));
#58546=CARTESIAN_POINT('Ctrl Pts',(-16.6995564402482,-17.3958177224365,
-20.5501102243653));
#58547=CARTESIAN_POINT('Ctrl Pts',(-16.6507112074467,-17.4642137899477,
-20.5542801172065));
#58548=CARTESIAN_POINT('Ctrl Pts',(-16.6018146060796,-17.5326817868506,
-20.5584543953561));
#58549=CARTESIAN_POINT('Ctrl Pts',(-16.556320811115,-17.6035292833675,-20.5626286735058));
#58550=CARTESIAN_POINT('Ctrl Pts',(-16.5144528430049,-17.6763784190149,
-20.5668029516555));
#58551=CARTESIAN_POINT('Ctrl Pts',(-16.4725619106312,-17.7492675118618,
-20.5709795193651));
#58552=CARTESIAN_POINT('Ctrl Pts',(-16.434300974443,-17.8241600201155,-20.5751560870748));
#58553=CARTESIAN_POINT('Ctrl Pts',(-16.3998462116972,-17.9006551029506,
-20.5793326547844));
#58554=CARTESIAN_POINT('Ctrl Pts',(-16.3653318275832,-17.9772825547571,
-20.5835164497295));
#58555=CARTESIAN_POINT('Ctrl Pts',(-16.3346369396098,-18.0555176912515,
-20.5877002446745));
#58556=CARTESIAN_POINT('Ctrl Pts',(-16.3078887870756,-18.1349416284485,
-20.5918840396196));
#58557=CARTESIAN_POINT('Ctrl Pts',(-16.2883209175697,-18.1930449773331,
-20.5949447352478));
#58558=CARTESIAN_POINT('Ctrl Pts',(-16.2708642209569,-18.2517841874754,
-20.598005430876));
#58559=CARTESIAN_POINT('Ctrl Pts',(-16.2555511525118,-18.3109919576289,
-20.6010661265042));
#58560=CARTESIAN_POINT('Ctrl Pts',(-16.2346154345157,-18.3919396255347,
-20.6052506477694));
#58561=CARTESIAN_POINT('Ctrl Pts',(-16.2176106157921,-18.4740647181832,
-20.6094351690346));
#58562=CARTESIAN_POINT('Ctrl Pts',(-16.2046649096203,-18.5569506352696,
-20.6136196902999));
#58563=CARTESIAN_POINT('Ctrl Pts',(-16.1917376309692,-18.6397185686836,
-20.6177982551227));
#58564=CARTESIAN_POINT('Ctrl Pts',(-16.1828580584881,-18.7232447247143,
-20.6219768199456));
#58565=CARTESIAN_POINT('Ctrl Pts',(-16.1781041153418,-18.8070992519429,
-20.6261553847685));
#58566=CARTESIAN_POINT('Ctrl Pts',(-16.1732647978195,-18.8924596928359,
-20.6304089909525));
#58567=CARTESIAN_POINT('Ctrl Pts',(-16.1727008779273,-18.9781599489881,
-20.6346625971366));
#58568=CARTESIAN_POINT('Ctrl Pts',(-16.1764397017154,-19.0637377314903,
-20.6389162033206));
#58569=CARTESIAN_POINT('Ctrl Pts',(-16.1801059175876,-19.1476535944188,
-20.6430872045204));
#58570=CARTESIAN_POINT('Ctrl Pts',(-16.1879092316882,-19.2314512172152,
-20.6472582057202));
#58571=CARTESIAN_POINT('Ctrl Pts',(-16.1998229036826,-19.3146933201762,
-20.65142920692));
#58572=CARTESIAN_POINT('Ctrl Pts',(-16.2117325790265,-19.3979074981112,
-20.6555988088842));
#58573=CARTESIAN_POINT('Ctrl Pts',(-16.2277498086426,-19.480566071281,-20.6597684108483));
#58574=CARTESIAN_POINT('Ctrl Pts',(-16.2477960843791,-19.5622377323235,
-20.6639380128125));
#58575=CARTESIAN_POINT('Ctrl Pts',(-16.2678416494881,-19.6439064981584,
-20.668107466967));
#58576=CARTESIAN_POINT('Ctrl Pts',(-16.2919158662461,-19.7245879748307,
-20.6722769211214));
#58577=CARTESIAN_POINT('Ctrl Pts',(-16.3198895960846,-19.8038632271131,
-20.6764463752759));
#58578=CARTESIAN_POINT('Ctrl Pts',(-16.3488485215244,-19.8859304427944,
-20.6807626717684));
#58579=CARTESIAN_POINT('Ctrl Pts',(-16.3819865838887,-19.9664900366014,
-20.6850789682609));
#58580=CARTESIAN_POINT('Ctrl Pts',(-16.4191057518191,-20.0450986322098,
-20.6893952647533));
#58581=CARTESIAN_POINT('Ctrl Pts',(-16.4550137144482,-20.1211422148332,
-20.6935707196945));
#58582=CARTESIAN_POINT('Ctrl Pts',(-16.4946467067841,-20.1953597704704,
-20.6977461746357));
#58583=CARTESIAN_POINT('Ctrl Pts',(-16.5377789910434,-20.2673757181192,
-20.7019216295769));
#58584=CARTESIAN_POINT('Ctrl Pts',(-16.5830936067771,-20.3430354020531,
-20.7063083468451));
#58585=CARTESIAN_POINT('Ctrl Pts',(-16.6322706296986,-20.4162643312086,
-20.7106950641132));
#58586=CARTESIAN_POINT('Ctrl Pts',(-16.6849987382266,-20.4866640770054,
-20.7150817813813));
#58587=CARTESIAN_POINT('Ctrl Pts',(-16.7377268467545,-20.5570638228022,
-20.7194684986494));
#58588=CARTESIAN_POINT('Ctrl Pts',(-16.7940056108791,-20.6246339879283,
-20.7238552159176));
#58589=CARTESIAN_POINT('Ctrl Pts',(-16.8534788452301,-20.689020491089,-20.7282419331857));
#58590=CARTESIAN_POINT('Ctrl Pts',(-16.9102137581221,-20.7504424515406,
-20.7324266731751));
#58591=CARTESIAN_POINT('Ctrl Pts',(-16.9700666644563,-20.8091961438448,
-20.7366114131645));
#58592=CARTESIAN_POINT('Ctrl Pts',(-17.0327566307066,-20.8649482477149,
-20.740796153154));
#58593=CARTESIAN_POINT('Ctrl Pts',(-17.0953573578707,-20.9206209885368,
-20.7449749361714));
#58594=CARTESIAN_POINT('Ctrl Pts',(-17.1607867823076,-20.9733003248918,
-20.7491537191888));
#58595=CARTESIAN_POINT('Ctrl Pts',(-17.2287256089521,-21.0226880517488,
-20.7533325022063));
#58596=CARTESIAN_POINT('Ctrl Pts',(-17.297880025795,-21.0729594446868,-20.7575860537755));
#58597=CARTESIAN_POINT('Ctrl Pts',(-17.3696342017319,-21.1198199228446,
-20.7618396053447));
#58598=CARTESIAN_POINT('Ctrl Pts',(-17.443614263699,-21.1629963029256,-20.7660931569139));
#58599=CARTESIAN_POINT('Ctrl Pts',(-17.5161623107921,-21.2053369278474,
-20.7702643734735));
#58600=CARTESIAN_POINT('Ctrl Pts',(-17.5908504241594,-21.244134565952,-20.774435590033));
#58601=CARTESIAN_POINT('Ctrl Pts',(-17.6672964146049,-21.2791749957631,
-20.7786068065926));
#58602=CARTESIAN_POINT('Ctrl Pts',(-17.7437167334923,-21.3142036585421,
-20.7827766224034));
#58603=CARTESIAN_POINT('Ctrl Pts',(-17.8218933392511,-21.3454774273092,
-20.7869464382142));
#58604=CARTESIAN_POINT('Ctrl Pts',(-17.9014210435259,-21.3728288417888,
-20.791116254025));
#58605=CARTESIAN_POINT('Ctrl Pts',(-17.9809458947181,-21.4001792750274,
-20.7952859202423));
#58606=CARTESIAN_POINT('Ctrl Pts',(-18.0618213127757,-21.4236074849553,
-20.7994555864596));
#58607=CARTESIAN_POINT('Ctrl Pts',(-18.1436251063839,-21.4429952800011,
-20.8036252526769));
#58608=CARTESIAN_POINT('Ctrl Pts',(-18.2283005878212,-21.463063675452,-20.807941293276));
#58609=CARTESIAN_POINT('Ctrl Pts',(-18.3139703255072,-21.4788025798654,
-20.8122573338752));
#58610=CARTESIAN_POINT('Ctrl Pts',(-18.4001544397717,-21.490138519056,-20.8165733744744));
#58611=CARTESIAN_POINT('Ctrl Pts',(-18.483535397029,-21.501105754366,-20.8207490349171));
#58612=CARTESIAN_POINT('Ctrl Pts',(-18.5673973100676,-21.5079520575122,
-20.8249246953598));
#58613=CARTESIAN_POINT('Ctrl Pts',(-18.6513021513138,-21.5106639220153,
-20.8291003558025));
#58614=CARTESIAN_POINT('Ctrl Pts',(-18.7394381464964,-21.513512540441,-20.8334865864799));
#58615=CARTESIAN_POINT('Ctrl Pts',(-18.827620929765,-21.5117987866347,-20.8378728171574));
#58616=CARTESIAN_POINT('Ctrl Pts',(-18.9153471676247,-21.5055687194189,
-20.8422590478348));
#58617=CARTESIAN_POINT('Ctrl Pts',(-19.0030734054844,-21.499338652203,-20.8466452785123));
#58618=CARTESIAN_POINT('Ctrl Pts',(-19.0903425315942,-21.4885924178744,
-20.8510315091897));
#58619=CARTESIAN_POINT('Ctrl Pts',(-19.1766642018011,-21.4734377653323,
-20.8554177398671));
#58620=CARTESIAN_POINT('Ctrl Pts',(-19.2590223589629,-21.4589789480642,
-20.8596025740416));
#58621=CARTESIAN_POINT('Ctrl Pts',(-19.3408245084339,-21.4404538839632,
-20.8637874082161));
#58622=CARTESIAN_POINT('Ctrl Pts',(-19.4216382989709,-21.4179184029056,
-20.8679722423906));
#58623=CARTESIAN_POINT('Ctrl Pts',(-19.5023371028523,-21.3954149866674,
-20.8721511221348));
#58624=CARTESIAN_POINT('Ctrl Pts',(-19.5820499018622,-21.3689126104334,
-20.8763300018789));
#58625=CARTESIAN_POINT('Ctrl Pts',(-19.6603531104247,-21.338518366744,-20.8805088816231));
#58626=CARTESIAN_POINT('Ctrl Pts',(-19.7400550610479,-21.3075811860814,
-20.8847624093283));
#58627=CARTESIAN_POINT('Ctrl Pts',(-19.8182960912148,-21.2726118104529,
-20.8890159370335));
#58628=CARTESIAN_POINT('Ctrl Pts',(-19.8946441530214,-21.2337767528961,
-20.8932694647388));
#58629=CARTESIAN_POINT('Ctrl Pts',(-19.9695166174632,-21.195692269843,-20.8974407834904));
#58630=CARTESIAN_POINT('Ctrl Pts',(-20.0425682056166,-21.1538904198174,
-20.901612102242));
#58631=CARTESIAN_POINT('Ctrl Pts',(-20.1134119104384,-21.1085766347016,
-20.9057834209936));
#58632=CARTESIAN_POINT('Ctrl Pts',(-20.1842318561761,-21.0632780466174,
-20.9099533407964));
#58633=CARTESIAN_POINT('Ctrl Pts',(-20.2528450019901,-21.0144701102459,
-20.9141232605992));
#58634=CARTESIAN_POINT('Ctrl Pts',(-20.3188912127324,-20.9624029058384,
-20.9182931804021));
#58635=CARTESIAN_POINT('Ctrl Pts',(-20.3849350802549,-20.9103375486967,
-20.9224629522624));
#58636=CARTESIAN_POINT('Ctrl Pts',(-20.448411833077,-20.8550134388734,-20.9266327241228));
#58637=CARTESIAN_POINT('Ctrl Pts',(-20.5089935615136,-20.7967216203496,
-20.9308024959832));
#58638=CARTESIAN_POINT('Ctrl Pts',(-20.5716986579763,-20.7363866943274,
-20.9351184168636));
#58639=CARTESIAN_POINT('Ctrl Pts',(-20.6313016391124,-20.6728725241964,
-20.9394343377441));
#58640=CARTESIAN_POINT('Ctrl Pts',(-20.687481020985,-20.6065428071378,-20.9437502586245));
#58641=CARTESIAN_POINT('Ctrl Pts',(-20.7418360778663,-20.5423670290593,
-20.9479260276902));
#58642=CARTESIAN_POINT('Ctrl Pts',(-20.79298623453,-20.4755561680757,-20.9521017967558));
#58643=CARTESIAN_POINT('Ctrl Pts',(-20.8406830326348,-20.4064712441326,
-20.9562775658215));
#58644=CARTESIAN_POINT('Ctrl Pts',(-20.8907811103752,-20.333908262383,-20.9606635626093));
#58645=CARTESIAN_POINT('Ctrl Pts',(-20.9370686806316,-20.2588367305564,
-20.9650495593971));
#58646=CARTESIAN_POINT('Ctrl Pts',(-20.9793120741947,-20.1817047163753,
-20.969435556185));
#58647=CARTESIAN_POINT('Ctrl Pts',(-21.0215554677577,-20.1045727021941,
-20.9738215529728));
#58648=CARTESIAN_POINT('Ctrl Pts',(-21.0597545011784,-20.025380760798,-20.9782075497606));
#58649=CARTESIAN_POINT('Ctrl Pts',(-21.0937343889893,-19.9445994224366,
-20.9825935465485));
#58650=CARTESIAN_POINT('Ctrl Pts',(-21.1297844964522,-19.8588964929525,
-20.9872467595436));
#58651=CARTESIAN_POINT('Ctrl Pts',(-21.1612011352353,-19.7711341998165,
-20.9918999725387));
#58652=CARTESIAN_POINT('Ctrl Pts',(-21.187770405969,-19.6818018873577,-20.9965531855338));
#58653=CARTESIAN_POINT('Ctrl Pts',(-21.2142564631891,-19.5927493588517,
-21.0011918249184));
#58654=CARTESIAN_POINT('Ctrl Pts',(-21.2359253189815,-19.5021368713044,
-21.005830464303));
#58655=CARTESIAN_POINT('Ctrl Pts',(-21.2526114126831,-19.410471975046,-21.0104691036876));
#58656=CARTESIAN_POINT('Ctrl Pts',(-21.269207206213,-19.3193031419175,-21.0150826401368));
#58657=CARTESIAN_POINT('Ctrl Pts',(-21.2808739033347,-19.2270935185721,
-21.019696176586));
#58658=CARTESIAN_POINT('Ctrl Pts',(-21.2874964963647,-19.1343612981233,
-21.0243097130352));
#58659=CARTESIAN_POINT('Ctrl Pts',(-21.2917935126354,-19.074192742048,-21.0273031690875));
#58660=CARTESIAN_POINT('Ctrl Pts',(-21.2939679585382,-19.0138045492422,
-21.0302966251399));
#58661=CARTESIAN_POINT('Ctrl Pts',(-21.29399964838,-18.9533417503911,-21.0332900811922));
#58662=CARTESIAN_POINT('Ctrl Pts',(-21.2904839170199,-18.9533393312605,
-21.0332901097715));
#58663=CARTESIAN_POINT('Ctrl Pts',(-21.2880301337774,-18.4391275099938,
-21.0587831909243));
#58664=CARTESIAN_POINT('Ctrl Pts',(-20.8878308621683,-17.0663417376224,
-21.1266682076376));
#58665=CARTESIAN_POINT('Ctrl Pts',(-18.9689508313882,-16.0899930897032,
-21.2211093015402));
#58666=CARTESIAN_POINT('Ctrl Pts',(-17.6030345805997,-16.6008609759918,
-21.29005731429));
#58667=CARTESIAN_POINT('Ctrl Pts',(-17.1763092963129,-16.9243021577153,
-21.3166133914793));
#58668=CARTESIAN_POINT('',(-21.2964370555865,-18.950145562236,-20.9667098902285));
#58669=CARTESIAN_POINT('Ctrl Pts',(-21.2964370555865,-18.950145562236,-20.9667098902285));
#58670=CARTESIAN_POINT('Ctrl Pts',(-21.2973788539875,-18.8345295300019,
-20.9724759609645));
#58671=CARTESIAN_POINT('Ctrl Pts',(-21.2376962631739,-17.8698878407826,
-21.0206339672611));
#58672=CARTESIAN_POINT('Ctrl Pts',(-20.0126665202556,-16.2082458119612,
-21.1111839091181));
#58673=CARTESIAN_POINT('Ctrl Pts',(-17.9939164803171,-16.3361984191612,
-21.1999086069035));
#58674=CARTESIAN_POINT('Ctrl Pts',(-17.2346906331956,-16.8707090898308,
-21.2462413691284));
#58675=CARTESIAN_POINT('Ctrl Pts',(-17.1724222329607,-16.9192441176791,
-21.2501821957929));
#58676=CARTESIAN_POINT('Ctrl Pts',(-17.1739275304995,-16.9211547578705,
-20.4499991767296));
#58677=CARTESIAN_POINT('Ctrl Pts',(-17.0385457733845,-17.0229919684527,
-20.4584344097234));
#58678=CARTESIAN_POINT('Ctrl Pts',(-16.286220291287,-17.716545158234,-20.5092615782776));
#58679=CARTESIAN_POINT('Ctrl Pts',(-15.8255862213472,-19.7912991220784,
-20.6024806823924));
#58680=CARTESIAN_POINT('Ctrl Pts',(-17.8654474230527,-21.8518086612915,
-20.7296564890738));
#58681=CARTESIAN_POINT('Ctrl Pts',(-20.5735369035609,-21.279131873543,-20.8510662250192));
#58682=CARTESIAN_POINT('Ctrl Pts',(-21.2904547875037,-19.6845342581055,
-20.9300840254041));
#58683=CARTESIAN_POINT('Ctrl Pts',(-21.2964370555865,-18.950145562236,-20.9667098902285));
#58684=CARTESIAN_POINT('Origin',(-18.734,-18.952,1.76670989022851));
#58685=CARTESIAN_POINT('',(-17.1744641548914,-16.9218650419685,-19.6501081133027));
#58686=CARTESIAN_POINT('',(-17.1744641548914,-16.9218650419685,-19.7167245499181));
#58687=CARTESIAN_POINT('',(-17.1744641548914,-16.9218650419685,1.76670989022851));
#58688=CARTESIAN_POINT('',(-21.2939995273704,-18.9535555909848,-20.2332901098006));
#58689=CARTESIAN_POINT('Ctrl Pts',(-17.1744641548914,-16.9218650419685,
-19.7167245499181));
#58690=CARTESIAN_POINT('Ctrl Pts',(-17.1080939778308,-16.9728501598607,
-19.7209062184222));
#58691=CARTESIAN_POINT('Ctrl Pts',(-17.0441148850582,-17.027179288429,-19.7250878869263));
#58692=CARTESIAN_POINT('Ctrl Pts',(-16.9828821694244,-17.0845990405271,
-19.7292695554304));
#58693=CARTESIAN_POINT('Ctrl Pts',(-16.9217270963244,-17.141945984895,-19.7334459216164));
#58694=CARTESIAN_POINT('Ctrl Pts',(-16.8633118156132,-17.2023754551086,
-19.7376222878024));
#58695=CARTESIAN_POINT('Ctrl Pts',(-16.807959606527,-17.2655930494953,-19.7417986539884));
#58696=CARTESIAN_POINT('Ctrl Pts',(-16.7526597112601,-17.3287508964237,
-19.745971073057));
#58697=CARTESIAN_POINT('Ctrl Pts',(-16.7004174362064,-17.3946912859582,
-19.7501434921256));
#58698=CARTESIAN_POINT('Ctrl Pts',(-16.6515191818487,-17.4630830640927,
-19.7543159111942));
#58699=CARTESIAN_POINT('Ctrl Pts',(-16.602645405779,-17.5314406055519,-19.7584862415651));
#58700=CARTESIAN_POINT('Ctrl Pts',(-16.5571125936733,-17.6022467254762,
-19.7626565719359));
#58701=CARTESIAN_POINT('Ctrl Pts',(-16.5151660691643,-17.6751382269908,
-19.7668269023067));
#58702=CARTESIAN_POINT('Ctrl Pts',(-16.4732279599042,-17.7480151051215,
-19.7709963960321));
#58703=CARTESIAN_POINT('Ctrl Pts',(-16.4348749381907,-17.8229761350483,
-19.7751658897574));
#58704=CARTESIAN_POINT('Ctrl Pts',(-16.4003075630717,-17.8996314287172,
-19.7793353834828));
#58705=CARTESIAN_POINT('Ctrl Pts',(-16.3657367535408,-17.9762943384071,
-19.7835052914647));
#58706=CARTESIAN_POINT('Ctrl Pts',(-16.3349525253485,-18.054651426181,-19.7876751994465));
#58707=CARTESIAN_POINT('Ctrl Pts',(-16.3081076999676,-18.1342918927617,
-19.7918451074284));
#58708=CARTESIAN_POINT('Ctrl Pts',(-16.2812344036413,-18.2140168240145,
-19.7960194379095));
#58709=CARTESIAN_POINT('Ctrl Pts',(-16.2583089990828,-18.2950274148578,
-19.8001937683907));
#58710=CARTESIAN_POINT('Ctrl Pts',(-16.2394345486869,-18.3768972186511,
-19.8043680988719));
#58711=CARTESIAN_POINT('Ctrl Pts',(-16.2205494936018,-18.4588130213379,
-19.8085447747182));
#58712=CARTESIAN_POINT('Ctrl Pts',(-16.2057200054997,-18.5415885452313,
-19.8127214505646));
#58713=CARTESIAN_POINT('Ctrl Pts',(-16.1949976382843,-18.6247890478577,
-19.8168981264109));
#58714=CARTESIAN_POINT('Ctrl Pts',(-16.1842568801908,-18.708132255007,-19.8210819660424));
#58715=CARTESIAN_POINT('Ctrl Pts',(-16.177637347357,-18.7919014377924,-19.825265805674));
#58716=CARTESIAN_POINT('Ctrl Pts',(-16.1751385264366,-18.8756589290556,
-19.8294496453056));
#58717=CARTESIAN_POINT('Ctrl Pts',(-16.1734340309011,-18.9327915826007,
-19.8323035256756));
#58718=CARTESIAN_POINT('Ctrl Pts',(-16.1736457572909,-18.9899187852792,
-19.8351574060456));
#58719=CARTESIAN_POINT('Ctrl Pts',(-16.1757597065439,-19.0469031134252,
-19.8380112864157));
#58720=CARTESIAN_POINT('Ctrl Pts',(-16.1788593810972,-19.1304589848034,
-19.8421959187327));
#58721=CARTESIAN_POINT('Ctrl Pts',(-16.1860627143182,-19.2140183314082,
-19.8463805510498));
#58722=CARTESIAN_POINT('Ctrl Pts',(-16.1973733531442,-19.2971452657373,
-19.8505651833669));
#58723=CARTESIAN_POINT('Ctrl Pts',(-16.2086678926685,-19.3801538791111,
-19.8547438593752));
#58724=CARTESIAN_POINT('Ctrl Pts',(-16.224058063826,-19.462730850823,-19.8589225353834));
#58725=CARTESIAN_POINT('Ctrl Pts',(-16.2434955344908,-19.5444419864245,
-19.8631012113916));
#58726=CARTESIAN_POINT('Ctrl Pts',(-16.26328142009,-19.6276177868711,-19.867354789796));
#58727=CARTESIAN_POINT('Ctrl Pts',(-16.2872611153603,-19.7098959227523,
-19.8716083682004));
#58728=CARTESIAN_POINT('Ctrl Pts',(-16.3153285555786,-19.7908256338122,
-19.8758619466048));
#58729=CARTESIAN_POINT('Ctrl Pts',(-16.3428518367464,-19.8701863156202,
-19.8800330585225));
#58730=CARTESIAN_POINT('Ctrl Pts',(-16.3743056169175,-19.9482499366746,
-19.8842041704402));
#58731=CARTESIAN_POINT('Ctrl Pts',(-16.4095391526147,-20.0246051318974,
-19.8883752823579));
#58732=CARTESIAN_POINT('Ctrl Pts',(-16.4447608654386,-20.1009347055702,
-19.8925449946281));
#58733=CARTESIAN_POINT('Ctrl Pts',(-16.483759622288,-20.1755565745853,-19.8967147068984));
#58734=CARTESIAN_POINT('Ctrl Pts',(-16.526336784863,-20.2480799082353,-19.9008844191686));
#58735=CARTESIAN_POINT('Ctrl Pts',(-16.5689124324897,-20.3206006614147,
-19.9050539830753));
#58736=CARTESIAN_POINT('Ctrl Pts',(-16.6150659990477,-20.3910226314022,
-19.909223546982));
#58737=CARTESIAN_POINT('Ctrl Pts',(-16.6645538721764,-20.4589813283634,
-19.9133931108887));
#58738=CARTESIAN_POINT('Ctrl Pts',(-16.7157817319262,-20.5293294434996,
-19.9177092760727));
#58739=CARTESIAN_POINT('Ctrl Pts',(-16.7705824262632,-20.5970374134405,
-19.9220254412568));
#58740=CARTESIAN_POINT('Ctrl Pts',(-16.8286393907572,-20.6617370993067,
-19.9263416064408));
#58741=CARTESIAN_POINT('Ctrl Pts',(-16.8848050972204,-20.7243291344967,
-19.9305171686474));
#58742=CARTESIAN_POINT('Ctrl Pts',(-16.9440178143264,-20.7841055699944,
-19.934692730854));
#58743=CARTESIAN_POINT('Ctrl Pts',(-17.0059537742783,-20.8407710930044,
-19.9388682930607));
#58744=CARTESIAN_POINT('Ctrl Pts',(-17.0710180723843,-20.9002987484136,
-19.9432547597334));
#58745=CARTESIAN_POINT('Ctrl Pts',(-17.1390875037942,-20.9563925860382,
-19.9476412264061));
#58746=CARTESIAN_POINT('Ctrl Pts',(-17.2097498583892,-21.0087599533732,
-19.9520276930789));
#58747=CARTESIAN_POINT('Ctrl Pts',(-17.2804122129843,-21.0611273207081,
-19.9564141597516));
#58748=CARTESIAN_POINT('Ctrl Pts',(-17.3536669653183,-21.1097679601685,
-19.9608006264243));
#58749=CARTESIAN_POINT('Ctrl Pts',(-17.4290716122084,-21.1544445288669,
-19.965187093097));
#58750=CARTESIAN_POINT('Ctrl Pts',(-17.5010067187011,-21.1970654263791,
-19.969371728398));
#58751=CARTESIAN_POINT('Ctrl Pts',(-17.5751659818923,-21.2362376725991,
-19.9735563636989));
#58752=CARTESIAN_POINT('Ctrl Pts',(-17.6511848628854,-21.2717222632969,
-19.9777409989998));
#58753=CARTESIAN_POINT('Ctrl Pts',(-17.7270955401342,-21.307156345943,-19.9819196779751));
#58754=CARTESIAN_POINT('Ctrl Pts',(-17.8048601642347,-21.338913006185,-19.9860983569504));
#58755=CARTESIAN_POINT('Ctrl Pts',(-17.8840874846205,-21.3667978623896,
-19.9902770359257));
#58756=CARTESIAN_POINT('Ctrl Pts',(-17.9647348763175,-21.3951825270456,
-19.9945306135862));
#58757=CARTESIAN_POINT('Ctrl Pts',(-18.04689750213,-21.4195549745919,-19.9987841912467));
#58758=CARTESIAN_POINT('Ctrl Pts',(-18.1301389338576,-21.4397604010028,
-20.0030377689073));
#58759=CARTESIAN_POINT('Ctrl Pts',(-18.2117665888522,-21.4595741108567,
-20.0072088837303));
#58760=CARTESIAN_POINT('Ctrl Pts',(-18.2944311264172,-21.4753808138487,
-20.0113799985533));
#58761=CARTESIAN_POINT('Ctrl Pts',(-18.377705058588,-21.4870845971534,-20.0155511133763));
#58762=CARTESIAN_POINT('Ctrl Pts',(-18.460951047014,-21.4987844530881,-20.0197208285227));
#58763=CARTESIAN_POINT('Ctrl Pts',(-18.5448055687472,-21.5063840596946,
-20.0238905436692));
#58764=CARTESIAN_POINT('Ctrl Pts',(-18.6288324774108,-21.5098388909766,
-20.0280602588157));
#58765=CARTESIAN_POINT('Ctrl Pts',(-18.7128563956359,-21.5132935993045,
-20.0322298255659));
#58766=CARTESIAN_POINT('Ctrl Pts',(-18.7970522289138,-21.5126038075458,
-20.0363993923161));
#58767=CARTESIAN_POINT('Ctrl Pts',(-18.8809816357491,-21.507777063586,-20.0405689590664));
#58768=CARTESIAN_POINT('Ctrl Pts',(-18.9678618598034,-21.5027806194017,
-20.0448851207924));
#58769=CARTESIAN_POINT('Ctrl Pts',(-19.0544560474151,-21.4933509339532,
-20.0492012825184));
#58770=CARTESIAN_POINT('Ctrl Pts',(-19.1402833032843,-21.4795549207628,
-20.0535174442444));
#58771=CARTESIAN_POINT('Ctrl Pts',(-19.2233147796995,-21.466208305725,-20.057693009185));
#58772=CARTESIAN_POINT('Ctrl Pts',(-19.3056280710303,-21.4487756011034,
-20.0618685741256));
#58773=CARTESIAN_POINT('Ctrl Pts',(-19.3867996160279,-21.4273691969712,
-20.0660441390663));
#58774=CARTESIAN_POINT('Ctrl Pts',(-19.472070890686,-21.4048816199976,-20.070430599185));
#58775=CARTESIAN_POINT('Ctrl Pts',(-19.5560814940463,-21.3780085540522,
-20.0748170593037));
#58776=CARTESIAN_POINT('Ctrl Pts',(-19.6383622324208,-21.3469381938937,
-20.0792035194224));
#58777=CARTESIAN_POINT('Ctrl Pts',(-19.7206429707954,-21.3158678337352,
-20.0835899795411));
#58778=CARTESIAN_POINT('Ctrl Pts',(-19.8011933431874,-21.2806004817501,
-20.0879764396598));
#58779=CARTESIAN_POINT('Ctrl Pts',(-19.8795742651246,-21.2413797420009,
-20.0923628997785));
#58780=CARTESIAN_POINT('Ctrl Pts',(-19.9543489008138,-21.2039635384947,
-20.0965475399847));
#58781=CARTESIAN_POINT('Ctrl Pts',(-20.0274276531195,-21.162810473499,-20.100732180191));
#58782=CARTESIAN_POINT('Ctrl Pts',(-20.0984122388012,-21.11809769923,-20.1049168203972));
#58783=CARTESIAN_POINT('Ctrl Pts',(-20.1692957874189,-21.0734485676151,
-20.1090955043278));
#58784=CARTESIAN_POINT('Ctrl Pts',(-20.2380907042344,-21.0252500340151,
-20.1132741882584));
#58785=CARTESIAN_POINT('Ctrl Pts',(-20.3044217681325,-20.9737258642496,
-20.117452872189));
#58786=CARTESIAN_POINT('Ctrl Pts',(-20.371941651073,-20.9212782521244,-20.1217064486169));
#58787=CARTESIAN_POINT('Ctrl Pts',(-20.4369080609029,-20.865384834865,-20.1259600250449));
#58788=CARTESIAN_POINT('Ctrl Pts',(-20.4989546028882,-20.8063287868509,
-20.1302136014728));
#58789=CARTESIAN_POINT('Ctrl Pts',(-20.5597983582893,-20.7484175540028,
-20.1343847213367));
#58790=CARTESIAN_POINT('Ctrl Pts',(-20.6178340917841,-20.6874655447192,
-20.1385558412007));
#58791=CARTESIAN_POINT('Ctrl Pts',(-20.6727497644134,-20.6237802938745,
-20.1427269610646));
#58792=CARTESIAN_POINT('Ctrl Pts',(-20.7276470096087,-20.5601164131724,
-20.1468966812728));
#58793=CARTESIAN_POINT('Ctrl Pts',(-20.7794259730566,-20.4937214605129,
-20.151066401481));
#58794=CARTESIAN_POINT('Ctrl Pts',(-20.827813137392,-20.4249380658006,-20.1552361216892));
#58795=CARTESIAN_POINT('Ctrl Pts',(-20.8761985798384,-20.3561571187907,
-20.1594056935151));
#58796=CARTESIAN_POINT('Ctrl Pts',(-20.921192199164,-20.2849882754667,-20.1635752653411));
#58797=CARTESIAN_POINT('Ctrl Pts',(-20.9625630757428,-20.2118041980546,
-20.167744837167));
#58798=CARTESIAN_POINT('Ctrl Pts',(-21.0053883717902,-20.1360472878725,
-20.1720609929414));
#58799=CARTESIAN_POINT('Ctrl Pts',(-21.044331197893,-20.0581312678785,-20.1763771487158));
#58800=CARTESIAN_POINT('Ctrl Pts',(-21.0791875194638,-19.9784967114177,
-20.1806933044902));
#58801=CARTESIAN_POINT('Ctrl Pts',(-21.1129085013345,-19.9014560108021,
-20.184868874489));
#58802=CARTESIAN_POINT('Ctrl Pts',(-21.1428049796707,-19.8228074643854,
-20.1890444444878));
#58803=CARTESIAN_POINT('Ctrl Pts',(-21.1687421906793,-19.7429680555664,
-20.1932200144866));
#58804=CARTESIAN_POINT('Ctrl Pts',(-21.1959893077345,-19.6590965199184,
-20.1976064631488));
#58805=CARTESIAN_POINT('Ctrl Pts',(-21.2188665683597,-19.5739112349382,
-20.201992911811));
#58806=CARTESIAN_POINT('Ctrl Pts',(-21.2372782494394,-19.4879085797817,
-20.2063793604732));
#58807=CARTESIAN_POINT('Ctrl Pts',(-21.2556899305191,-19.4019059246253,
-20.2107658091355));
#58808=CARTESIAN_POINT('Ctrl Pts',(-21.2696360151318,-19.3150864842148,
-20.2151522577977));
#58809=CARTESIAN_POINT('Ctrl Pts',(-21.2790836671994,-19.2279513126528,
-20.2195387064599));
#58810=CARTESIAN_POINT('Ctrl Pts',(-21.2889563823072,-19.136895808223,-20.2241225075637));
#58811=CARTESIAN_POINT('Ctrl Pts',(-21.2939437779019,-19.0453011468624,
-20.2287063086676));
#58812=CARTESIAN_POINT('Ctrl Pts',(-21.2939995273701,-18.9535555915677,
-20.2332901097715));
#58813=CARTESIAN_POINT('Ctrl Pts',(-21.2939995273704,-18.9535555909848,
-20.2332901098006));
#58814=CARTESIAN_POINT('Ctrl Pts',(-21.294049723898,-18.870948345104,-20.2374173417263));
#58815=CARTESIAN_POINT('Ctrl Pts',(-21.2900972917066,-18.7881812203374,
-20.241544573652));
#58816=CARTESIAN_POINT('Ctrl Pts',(-21.2821221997477,-18.7056805830778,
-20.2456718055777));
#58817=CARTESIAN_POINT('Ctrl Pts',(-21.2739869562085,-18.6215232116386,
-20.2498819183928));
#58818=CARTESIAN_POINT('Ctrl Pts',(-21.2616656480612,-18.537643639815,-20.254092031208));
#58819=CARTESIAN_POINT('Ctrl Pts',(-21.2451929664636,-18.4544963465625,
-20.2583021440231));
#58820=CARTESIAN_POINT('Ctrl Pts',(-21.229080068103,-18.3731650904946,-20.2624203028958));
#58821=CARTESIAN_POINT('Ctrl Pts',(-21.2089953895162,-18.2925349412607,
-20.2665384617684));
#58822=CARTESIAN_POINT('Ctrl Pts',(-21.1850236976428,-18.2130258234598,
-20.270656620641));
#58823=CARTESIAN_POINT('Ctrl Pts',(-21.1610629749352,-18.1335530881012,
-20.2747728950923));
#58824=CARTESIAN_POINT('Ctrl Pts',(-21.1332189046361,-18.055200818656,-20.2788891695437));
#58825=CARTESIAN_POINT('Ctrl Pts',(-21.1016267121137,-17.9783759698499,
-20.283005443995));
#58826=CARTESIAN_POINT('Ctrl Pts',(-21.0700389130291,-17.9015618048605,
-20.2871211460075));
#58827=CARTESIAN_POINT('Ctrl Pts',(-21.0347042074052,-17.8262750760015,
-20.2912368480201));
#58828=CARTESIAN_POINT('Ctrl Pts',(-20.9958062193322,-17.752903412485,-20.2953525500326));
#58829=CARTESIAN_POINT('Ctrl Pts',(-20.9553538853537,-17.6765998506772,
-20.299632713625));
#58830=CARTESIAN_POINT('Ctrl Pts',(-20.9110477424172,-17.6023681210458,
-20.3039128772174));
#58831=CARTESIAN_POINT('Ctrl Pts',(-20.8631463424907,-17.5306148121433,
-20.3081930408098));
#58832=CARTESIAN_POINT('Ctrl Pts',(-20.817026382064,-17.4615299884816,-20.3123140263301));
#58833=CARTESIAN_POINT('Ctrl Pts',(-20.767574190865,-17.394742855338,-20.3164350118505));
#58834=CARTESIAN_POINT('Ctrl Pts',(-20.7150628530422,-17.3305839607626,
-20.3205559973708));
#58835=CARTESIAN_POINT('Ctrl Pts',(-20.6625158707606,-17.2663815154195,
-20.3246797801975));
#58836=CARTESIAN_POINT('Ctrl Pts',(-20.6069059305284,-17.204811205117,-20.3288035630242));
#58837=CARTESIAN_POINT('Ctrl Pts',(-20.5485433980296,-17.1461671570527,
-20.3329273458509));
#58838=CARTESIAN_POINT('Ctrl Pts',(-20.4900913111083,-17.0874331225942,
-20.3370574564186));
#58839=CARTESIAN_POINT('Ctrl Pts',(-20.4288785613994,-17.031634616857,-20.3411875669862));
#58840=CARTESIAN_POINT('Ctrl Pts',(-20.3652483132487,-16.9790253573542,
-20.3453176775539));
#58841=CARTESIAN_POINT('Ctrl Pts',(-20.3580748979454,-16.9730944034733,
-20.3457832894164));
#58842=CARTESIAN_POINT('Ctrl Pts',(-20.3508707868094,-16.9672039368768,
-20.3462489012788));
#58843=CARTESIAN_POINT('Ctrl Pts',(-20.3436364930174,-16.961354285578,-20.3467145131413));
#58844=CARTESIAN_POINT('Ctrl Pts',(-20.2786189220457,-16.9087810656599,
-20.3508991582751));
#58845=CARTESIAN_POINT('Ctrl Pts',(-20.2109019646558,-16.8592987216113,
-20.3550838034089));
#58846=CARTESIAN_POINT('Ctrl Pts',(-20.1408117772448,-16.813196450488,-20.3592684485427));
#58847=CARTESIAN_POINT('Ctrl Pts',(-20.0708213560678,-16.7671598012461,
-20.3634471372609));
#58848=CARTESIAN_POINT('Ctrl Pts',(-19.9984647957972,-16.724493919034,-20.3676258259791));
#58849=CARTESIAN_POINT('Ctrl Pts',(-19.9241011351325,-16.6854477089297,
-20.3718045146973));
#58850=CARTESIAN_POINT('Ctrl Pts',(-19.8484047994816,-16.6457017496864,
-20.3760580899108));
#58851=CARTESIAN_POINT('Ctrl Pts',(-19.7706290892635,-16.6097067834814,
-20.3803116651244));
#58852=CARTESIAN_POINT('Ctrl Pts',(-19.6911834645766,-16.5776790833712,
-20.384565240338));
#58853=CARTESIAN_POINT('Ctrl Pts',(-19.6132778070226,-16.5462722054359,
-20.3887363646167));
#58854=CARTESIAN_POINT('Ctrl Pts',(-19.5337668426417,-16.5186803435126,
-20.3929074888954));
#58855=CARTESIAN_POINT('Ctrl Pts',(-19.4530597028474,-16.4950602075466,
-20.3970786131741));
#58856=CARTESIAN_POINT('Ctrl Pts',(-19.3723796478629,-16.47144799835,-20.4012483376496));
#58857=CARTESIAN_POINT('Ctrl Pts',(-19.2905046558528,-16.4518049970839,
-20.4054180621252));
#58858=CARTESIAN_POINT('Ctrl Pts',(-19.2078598549769,-16.4362383185522,
-20.4095877866007));
#58859=CARTESIAN_POINT('Ctrl Pts',(-19.1252179980804,-16.4206721945378,
-20.4137573625421));
#58860=CARTESIAN_POINT('Ctrl Pts',(-19.0418068390792,-16.4091821888638,
-20.4179269384834));
#58861=CARTESIAN_POINT('Ctrl Pts',(-18.9580612068526,-16.4018242069254,
-20.4220965144247));
#58862=CARTESIAN_POINT('Ctrl Pts',(-18.8713716361879,-16.3942075673677,
-20.4264126648745));
#58863=CARTESIAN_POINT('Ctrl Pts',(-18.7843241636749,-16.3910189213341,
-20.4307288153244));
#58864=CARTESIAN_POINT('Ctrl Pts',(-18.6974043010312,-16.3922615846894,
-20.4350449657742));
#58865=CARTESIAN_POINT('Ctrl Pts',(-18.613315412911,-16.3934637745764,-20.4392205394722));
#58866=CARTESIAN_POINT('Ctrl Pts',(-18.5293464168604,-16.3988129730352,
-20.4433961131702));
#58867=CARTESIAN_POINT('Ctrl Pts',(-18.4459326746173,-16.4082592081647,
-20.4475716868682));
#58868=CARTESIAN_POINT('Ctrl Pts',(-18.3583065652387,-16.4181824751278,
-20.4519581256939));
#58869=CARTESIAN_POINT('Ctrl Pts',(-18.2712938422192,-16.432627374356,-20.4563445645197));
#58870=CARTESIAN_POINT('Ctrl Pts',(-18.1853859701636,-16.4514755257613,
-20.4607310033455));
#58871=CARTESIAN_POINT('Ctrl Pts',(-18.099478098108,-16.4703236771666,-20.4651174421712));
#58872=CARTESIAN_POINT('Ctrl Pts',(-18.0146756164478,-16.4935748539843,
-20.469503880997));
#58873=CARTESIAN_POINT('Ctrl Pts',(-17.9314482086937,-16.5210514974045,
-20.4738903198228));
#58874=CARTESIAN_POINT('Ctrl Pts',(-17.852064997737,-16.547259020141,-20.4780741531062));
#58875=CARTESIAN_POINT('Ctrl Pts',(-17.7738191753082,-16.5774078021578,
-20.4822579863897));
#58876=CARTESIAN_POINT('Ctrl Pts',(-17.6971302056129,-16.6113802039871,
-20.4864418196731));
#58877=CARTESIAN_POINT('Ctrl Pts',(-17.6205369308216,-16.6453102139868,
-20.490620432238));
#58878=CARTESIAN_POINT('Ctrl Pts',(-17.545497070241,-16.6830541908193,-20.4947990448029));
#58879=CARTESIAN_POINT('Ctrl Pts',(-17.4724142317339,-16.7244449839996,
-20.4989776573678));
#58880=CARTESIAN_POINT('Ctrl Pts',(-17.3994143757936,-16.7657887796313,
-20.5031515252895));
#58881=CARTESIAN_POINT('Ctrl Pts',(-17.3283675238019,-16.8107709366666,
-20.5073253932112));
#58882=CARTESIAN_POINT('Ctrl Pts',(-17.2596551356225,-16.85917721226,-20.5114992611328));
#58883=CARTESIAN_POINT('Ctrl Pts',(-17.2308389306407,-16.879477556883,-20.5132496737845));
#58884=CARTESIAN_POINT('Ctrl Pts',(-17.2024330111304,-16.9003795571347,
-20.5150000864362));
#58885=CARTESIAN_POINT('Ctrl Pts',(-17.1744641548914,-16.9218650419685,
-20.5167504990879));
#58886=CARTESIAN_POINT('',(-21.2937660523048,-18.9509923322678,-20.1667099325986));
#58887=CARTESIAN_POINT('Ctrl Pts',(-21.2901593135592,-18.9509805599729,
-20.1667105863666));
#58888=CARTESIAN_POINT('Ctrl Pts',(-21.2914430747328,-18.5861666271369,
-20.1847914783605));
#58889=CARTESIAN_POINT('Ctrl Pts',(-21.0477247281039,-17.3676608534593,
-20.2452643059147));
#58890=CARTESIAN_POINT('Ctrl Pts',(-19.3278236160818,-16.0727555198283,
-20.3396938360357));
#58891=CARTESIAN_POINT('Ctrl Pts',(-17.7189175814815,-16.5112009519086,
-20.4160424741629));
#58892=CARTESIAN_POINT('Ctrl Pts',(-17.1739275304995,-16.9211547578705,
-20.4499991767296));
#58893=CARTESIAN_POINT('Ctrl Pts',(-17.1744641548914,-16.9218650419685,
-19.6501081133027));
#58894=CARTESIAN_POINT('Ctrl Pts',(-17.1077737209788,-16.9730961789927,
-19.6542777804462));
#58895=CARTESIAN_POINT('Ctrl Pts',(-17.0436133363582,-17.0276146696201,
-19.6584474475896));
#58896=CARTESIAN_POINT('Ctrl Pts',(-16.9823134737079,-17.0851324863272,
-19.6626171147331));
#58897=CARTESIAN_POINT('Ctrl Pts',(-16.9209516901765,-17.1427084035543,
-19.6667909937859));
#58898=CARTESIAN_POINT('Ctrl Pts',(-16.862456536847,-17.2032893833971,-19.6709648728387));
#58899=CARTESIAN_POINT('Ctrl Pts',(-16.8071223186683,-17.2665497927302,
-19.6751387518915));
#58900=CARTESIAN_POINT('Ctrl Pts',(-16.7517611351814,-17.3298410299397,
-19.6793146649467));
#58901=CARTESIAN_POINT('Ctrl Pts',(-16.6995642411243,-17.3958139365116,
-19.6834905780019));
#58902=CARTESIAN_POINT('Ctrl Pts',(-16.6507846855712,-17.4641109067779,
-19.6876664910572));
#58903=CARTESIAN_POINT('Ctrl Pts',(-16.6019171798243,-17.5325310173988,
-19.6918499333398));
#58904=CARTESIAN_POINT('Ctrl Pts',(-16.5564795739258,-17.6032831769332,
-19.6960333756223));
#58905=CARTESIAN_POINT('Ctrl Pts',(-16.5146806856349,-17.6759820609075,
-19.7002168179049));
#58906=CARTESIAN_POINT('Ctrl Pts',(-16.4746040303209,-17.7456855442744,
-19.7042278904774));
#58907=CARTESIAN_POINT('Ctrl Pts',(-16.4378722519963,-17.817178139003,-19.7082389630498));
#58908=CARTESIAN_POINT('Ctrl Pts',(-16.4046276535563,-17.8901033611394,
-19.7122500356223));
#58909=CARTESIAN_POINT('Ctrl Pts',(-16.3699445411289,-17.9661841019766,
-19.7164346697438));
#58910=CARTESIAN_POINT('Ctrl Pts',(-16.3389281684892,-18.0441074153348,
-19.7206193038652));
#58911=CARTESIAN_POINT('Ctrl Pts',(-16.3117771822314,-18.1234852921757,
-19.7248039379867));
#58912=CARTESIAN_POINT('Ctrl Pts',(-16.2846648420429,-18.2027501844311,
-19.7289826157992));
#58913=CARTESIAN_POINT('Ctrl Pts',(-16.2614071073441,-18.2834650961696,
-19.7331612936118));
#58914=CARTESIAN_POINT('Ctrl Pts',(-16.2421554012958,-18.3652202321922,
-19.7373399714244));
#58915=CARTESIAN_POINT('Ctrl Pts',(-16.2225586206672,-18.4484407770037,
-19.7415935493777));
#58916=CARTESIAN_POINT('Ctrl Pts',(-16.207113098083,-18.5327387664133,-19.745847127331));
#58917=CARTESIAN_POINT('Ctrl Pts',(-16.1959260745188,-18.617663719001,-19.7501007052843));
#58918=CARTESIAN_POINT('Ctrl Pts',(-16.1849559341181,-18.7009422289687,
-19.7542718189934));
#58919=CARTESIAN_POINT('Ctrl Pts',(-16.1780807097886,-18.7848231320472,
-19.7584429327025));
#58920=CARTESIAN_POINT('Ctrl Pts',(-16.1753500450965,-18.8688711345423,
-19.7626140464116));
#58921=CARTESIAN_POINT('Ctrl Pts',(-16.1726202967043,-18.9528909339471,
-19.7667837604647));
#58922=CARTESIAN_POINT('Ctrl Pts',(-16.1740323608325,-19.0370772620014,
-19.7709534745177));
#58923=CARTESIAN_POINT('Ctrl Pts',(-16.1795838629395,-19.1209917120005,
-19.7751231885707));
#58924=CARTESIAN_POINT('Ctrl Pts',(-16.1851351675026,-19.2049031760004,
-19.7792927542493));
#58925=CARTESIAN_POINT('Ctrl Pts',(-16.1948255859618,-19.2885423222071,
-19.7834623199278));
#58926=CARTESIAN_POINT('Ctrl Pts',(-16.2086007337952,-19.3714741306116,
-19.7876318856064));
#58927=CARTESIAN_POINT('Ctrl Pts',(-16.2228602007955,-19.457321730907,-19.7919480486645));
#58928=CARTESIAN_POINT('Ctrl Pts',(-16.2414968944622,-19.5424108074415,
-19.7962642117226));
#58929=CARTESIAN_POINT('Ctrl Pts',(-16.26439285385,-19.6262703787688,-19.8005803747807));
#58930=CARTESIAN_POINT('Ctrl Pts',(-16.2865429767612,-19.7073982223639,
-19.8047559387142));
#58931=CARTESIAN_POINT('Ctrl Pts',(-16.3126789433259,-19.7873750001408,
-19.8089315026477));
#58932=CARTESIAN_POINT('Ctrl Pts',(-16.34264370885,-19.8657916002993,-19.8131070665811));
#58933=CARTESIAN_POINT('Ctrl Pts',(-16.3741219297554,-19.9481688530246,
-19.8174935292016));
#58934=CARTESIAN_POINT('Ctrl Pts',(-16.4098256651424,-20.0288236423437,
-19.821879991822));
#58935=CARTESIAN_POINT('Ctrl Pts',(-16.4495176194985,-20.1073095919183,
-19.8262664544424));
#58936=CARTESIAN_POINT('Ctrl Pts',(-16.4892095738547,-20.1857955414929,
-19.8306529170629));
#58937=CARTESIAN_POINT('Ctrl Pts',(-16.532889392945,-20.2621121855376,-19.8350393796833));
#58938=CARTESIAN_POINT('Ctrl Pts',(-16.5802679097415,-20.3358490103298,
-19.8394258423038));
#58939=CARTESIAN_POINT('Ctrl Pts',(-16.62546646493,-20.4061930854538,-19.8436104767381));
#58940=CARTESIAN_POINT('Ctrl Pts',(-16.6741990691197,-20.4744513619179,
-19.8477951111724));
#58941=CARTESIAN_POINT('Ctrl Pts',(-16.7262469917103,-20.5402467874054,
-19.8519797456066));
#58942=CARTESIAN_POINT('Ctrl Pts',(-16.7782208304952,-20.6059485612105,
-19.8561584237293));
#58943=CARTESIAN_POINT('Ctrl Pts',(-16.8335003313994,-20.6691940894861,
-19.860337101852));
#58944=CARTESIAN_POINT('Ctrl Pts',(-16.8918228839615,-20.7296342349157,
-19.8645157799747));
#58945=CARTESIAN_POINT('Ctrl Pts',(-16.9511908256725,-20.7911577257993,
-19.8687693578502));
#58946=CARTESIAN_POINT('Ctrl Pts',(-17.0137117247795,-20.849773866074,-19.8730229357256));
#58947=CARTESIAN_POINT('Ctrl Pts',(-17.0790648452578,-20.9051486460581,
-19.877276513601));
#58948=CARTESIAN_POINT('Ctrl Pts',(-17.1431509686188,-20.9594498784273,
-19.8814476276115));
#58949=CARTESIAN_POINT('Ctrl Pts',(-17.2099601099664,-21.0106339979947,
-19.8856187416219));
#58950=CARTESIAN_POINT('Ctrl Pts',(-17.2791531272801,-21.0584236461208,
-19.8897898556323));
#58951=CARTESIAN_POINT('Ctrl Pts',(-17.3483229261688,-21.1061972579417,
-19.8939595699827));
#58952=CARTESIAN_POINT('Ctrl Pts',(-17.4198746341319,-21.150578399273,-19.8981292843331));
#58953=CARTESIAN_POINT('Ctrl Pts',(-17.4934383351829,-21.1913317654573,
-19.9022989986835));
#58954=CARTESIAN_POINT('Ctrl Pts',(-17.5669994184791,-21.2320836814384,
-19.9064685646552));
#58955=CARTESIAN_POINT('Ctrl Pts',(-17.6425719496892,-21.2692078567604,
-19.9106381306269));
#58956=CARTESIAN_POINT('Ctrl Pts',(-17.7197607084836,-21.302514552081,-19.9148076965986));
#58957=CARTESIAN_POINT('Ctrl Pts',(-17.7996633275439,-21.3369922691724,
-19.9191238592974));
#58958=CARTESIAN_POINT('Ctrl Pts',(-17.8812974576163,-21.367378857563,-19.9234400219963));
#58959=CARTESIAN_POINT('Ctrl Pts',(-17.9642032279854,-21.3935185704385,
-19.9277561846952));
#58960=CARTESIAN_POINT('Ctrl Pts',(-18.0444083527598,-21.4188067852806,
-19.9319317489083));
#58961=CARTESIAN_POINT('Ctrl Pts',(-18.1258030751317,-21.4401204858059,
-19.9361073131214));
#58962=CARTESIAN_POINT('Ctrl Pts',(-18.2079583914654,-21.4573702772425,
-19.9402828773344));
#58963=CARTESIAN_POINT('Ctrl Pts',(-18.2942631756871,-21.475491314252,-19.9446693392762));
#58964=CARTESIAN_POINT('Ctrl Pts',(-18.38140683144,-21.4891270269169,-19.949055801218));
#58965=CARTESIAN_POINT('Ctrl Pts',(-18.4688855835814,-21.498235328128,-19.9534422631598));
#58966=CARTESIAN_POINT('Ctrl Pts',(-18.5563643357229,-21.5073436293391,
-19.9578287251016));
#58967=CARTESIAN_POINT('Ctrl Pts',(-18.6441776008613,-21.5119245648311,
-19.9622151870434));
#58968=CARTESIAN_POINT('Ctrl Pts',(-18.7318236815561,-21.5119990749291,
-19.9666016489852));
#58969=CARTESIAN_POINT('Ctrl Pts',(-18.8154370559313,-21.5120701567239,
-19.9707862843005));
#58970=CARTESIAN_POINT('Ctrl Pts',(-18.8992095169516,-21.508040657495,-19.9749709196158));
#58971=CARTESIAN_POINT('Ctrl Pts',(-18.9827056283928,-21.4998904039236,
-19.9791555549311));
#58972=CARTESIAN_POINT('Ctrl Pts',(-19.0660828935662,-21.4917517512183,
-19.9833342339415));
#58973=CARTESIAN_POINT('Ctrl Pts',(-19.149184136535,-21.4795040389676,-19.987512912952));
#58974=CARTESIAN_POINT('Ctrl Pts',(-19.2315736418543,-21.4631790997322,
-19.9916915919625));
#58975=CARTESIAN_POINT('Ctrl Pts',(-19.3154398966918,-21.446561552281,-19.9959451696169));
#58976=CARTESIAN_POINT('Ctrl Pts',(-19.3985681653821,-21.4257191734759,
-20.0001987472712));
#58977=CARTESIAN_POINT('Ctrl Pts',(-19.4805039905309,-21.400740858507,-20.0044523249255));
#58978=CARTESIAN_POINT('Ctrl Pts',(-19.560851352111,-21.3762467901208,-20.0086234398338));
#58979=CARTESIAN_POINT('Ctrl Pts',(-19.6400516322992,-21.3477758589918,
-20.0127945547421));
#58980=CARTESIAN_POINT('Ctrl Pts',(-19.7176880451009,-21.315463101029,-20.0169656696504));
#58981=CARTESIAN_POINT('Ctrl Pts',(-19.7952984062491,-21.2831611859264,
-20.0211353849005));
#58982=CARTESIAN_POINT('Ctrl Pts',(-19.8713455178527,-21.247020180909,-20.0253051001507));
#58983=CARTESIAN_POINT('Ctrl Pts',(-19.9454312973038,-21.207223760941,-20.0294748154008));
#58984=CARTESIAN_POINT('Ctrl Pts',(-20.0195144404333,-21.1674287571174,
-20.0336443822728));
#58985=CARTESIAN_POINT('Ctrl Pts',(-20.0916359853166,-21.1239788154148,
-20.0378139491447));
#58986=CARTESIAN_POINT('Ctrl Pts',(-20.1614224658083,-21.0771035513842,
-20.0419835160167));
#58987=CARTESIAN_POINT('Ctrl Pts',(-20.2336625183512,-21.0285802340787,
-20.0462996776542));
#58988=CARTESIAN_POINT('Ctrl Pts',(-20.3033998142158,-20.9763865417844,
-20.0506158392917));
#58989=CARTESIAN_POINT('Ctrl Pts',(-20.3702544760718,-20.9208248498876,
-20.0549320009292));
#58990=CARTESIAN_POINT('Ctrl Pts',(-20.4349313850112,-20.8670730487782,
-20.0591075660348));
#58991=CARTESIAN_POINT('Ctrl Pts',(-20.4969102618753,-20.8101696539258,
-20.0632831311405));
#58992=CARTESIAN_POINT('Ctrl Pts',(-20.555883728143,-20.7504270018902,-20.0674586962461));
#58993=CARTESIAN_POINT('Ctrl Pts',(-20.6178357606472,-20.6876669344389,
-20.0718451561495));
#58994=CARTESIAN_POINT('Ctrl Pts',(-20.6764704135552,-20.6217736908107,
-20.0762316160529));
#58995=CARTESIAN_POINT('Ctrl Pts',(-20.7314796147868,-20.5531480845041,
-20.0806180759564));
#58996=CARTESIAN_POINT('Ctrl Pts',(-20.7864888160183,-20.4845224781975,
-20.0850045358598));
#58997=CARTESIAN_POINT('Ctrl Pts',(-20.8378722882511,-20.4131650245059,
-20.0893909957632));
#58998=CARTESIAN_POINT('Ctrl Pts',(-20.8853760799667,-20.3395089053938,
-20.0937774556666));
#58999=CARTESIAN_POINT('Ctrl Pts',(-20.93172083375,-20.2676499109516,-20.0980568909888));
#59000=CARTESIAN_POINT('Ctrl Pts',(-20.9745398784111,-20.1933453659579,
-20.1023363263109));
#59001=CARTESIAN_POINT('Ctrl Pts',(-21.0135728621542,-20.1169667661055,
-20.1066157616331));
#59002=CARTESIAN_POINT('Ctrl Pts',(-21.0525424988234,-20.0407121219527,
-20.1108882518109));
#59003=CARTESIAN_POINT('Ctrl Pts',(-21.0877380945303,-19.9623904961899,
-20.1151607419887));
#59004=CARTESIAN_POINT('Ctrl Pts',(-21.1189429603293,-19.8824015670536,
-20.1194332321666));
#59005=CARTESIAN_POINT('Ctrl Pts',(-21.1500944336146,-19.8025495015083,
-20.1236984119784));
#59006=CARTESIAN_POINT('Ctrl Pts',(-21.1772686126578,-19.7210362114978,
-20.1279635917902));
#59007=CARTESIAN_POINT('Ctrl Pts',(-21.2002957121622,-19.6382838043918,
-20.132228771602));
#59008=CARTESIAN_POINT('Ctrl Pts',(-21.2232995983466,-19.5556148189128,
-20.1364896517415));
#59009=CARTESIAN_POINT('Ctrl Pts',(-21.242164599727,-19.4717096138904,-20.1407505318809));
#59010=CARTESIAN_POINT('Ctrl Pts',(-21.2567699769455,-19.3870076360505,
-20.1450114120204));
#59011=CARTESIAN_POINT('Ctrl Pts',(-21.2713627640963,-19.3023786726647,
-20.1492686192133));
#59012=CARTESIAN_POINT('Ctrl Pts',(-21.2817031592285,-19.2169547278876,
-20.1535258264062));
#59013=CARTESIAN_POINT('Ctrl Pts',(-21.2877212407691,-19.1311865632376,
-20.1577830335991));
#59014=CARTESIAN_POINT('Ctrl Pts',(-21.2919276409326,-19.0712380199392,
-20.1607586524755));
#59015=CARTESIAN_POINT('Ctrl Pts',(-21.2940234518483,-19.0111215769093,
-20.163734271352));
#59016=CARTESIAN_POINT('Ctrl Pts',(-21.293999801981,-18.9509930952203,-20.1667098902285));
#59017=CARTESIAN_POINT('Origin',(-18.734,-18.952,1.76670989022851));
#59018=CARTESIAN_POINT('',(-17.1744641548914,-16.9218650419685,-18.8501886385061));
#59019=CARTESIAN_POINT('',(-17.1746506085037,-16.9221163620956,-18.9165758982197));
#59020=CARTESIAN_POINT('',(-17.1744641548914,-16.9218650419685,1.76670989022851));
#59021=CARTESIAN_POINT('',(-21.2939990581247,-18.9498040034555,-19.4332901097715));
#59022=CARTESIAN_POINT('Ctrl Pts',(-17.1746506085039,-16.9221163620955,
-18.9165758982197));
#59023=CARTESIAN_POINT('Ctrl Pts',(-17.0075187310044,-17.0478570694681,
-18.926977478695));
#59024=CARTESIAN_POINT('Ctrl Pts',(-16.2393387966466,-17.7870024615573,
-18.9797709947307));
#59025=CARTESIAN_POINT('Ctrl Pts',(-15.867552077141,-19.9250196648857,-19.074956446327));
#59026=CARTESIAN_POINT('Ctrl Pts',(-18.0006016646393,-21.8889061712022,
-19.2021322530084));
#59027=CARTESIAN_POINT('Ctrl Pts',(-20.6359183918341,-21.202775782827,-19.3215765970986));
#59028=CARTESIAN_POINT('Ctrl Pts',(-21.2889868109407,-19.6455867711505,
-19.3986290056282));
#59029=CARTESIAN_POINT('Ctrl Pts',(-21.2953147898194,-18.9498155448408,
-19.4332894785973));
#59030=CARTESIAN_POINT('Ctrl Pts',(-21.2939990581247,-18.9498040034555,
-19.4332901097715));
#59031=CARTESIAN_POINT('Ctrl Pts',(-21.2938905873826,-18.8233534412897,
-19.4395926510315));
#59032=CARTESIAN_POINT('Ctrl Pts',(-21.2844099378408,-18.6972910724131,
-19.4458951922915));
#59033=CARTESIAN_POINT('Ctrl Pts',(-21.2657470116111,-18.5727150554023,
-19.4521977335515));
#59034=CARTESIAN_POINT('Ctrl Pts',(-21.2615163488077,-18.544475158032,-19.4536264444915));
#59035=CARTESIAN_POINT('Ctrl Pts',(-21.25681399964,-18.5163115073431,-19.4550551554314));
#59036=CARTESIAN_POINT('Ctrl Pts',(-21.2516424693647,-18.4882367021301,
-19.4564838663713));
#59037=CARTESIAN_POINT('Ctrl Pts',(-21.2364952751732,-18.4060067810402,
-19.4606685004929));
#59038=CARTESIAN_POINT('Ctrl Pts',(-21.2172870302558,-18.3243667083798,
-19.4648531346144));
#59039=CARTESIAN_POINT('Ctrl Pts',(-21.1940771445919,-18.2437483196936,
-19.469037768736));
#59040=CARTESIAN_POINT('Ctrl Pts',(-21.1709002953281,-18.1632446813081,
-19.4732164465487));
#59041=CARTESIAN_POINT('Ctrl Pts',(-21.1437332452338,-18.0837602766129,
-19.4773951243614));
#59042=CARTESIAN_POINT('Ctrl Pts',(-21.112686592475,-18.0057177509962,-19.4815738021741));
#59043=CARTESIAN_POINT('Ctrl Pts',(-21.0810834482228,-17.9262763627721,
-19.4858273801273));
#59044=CARTESIAN_POINT('Ctrl Pts',(-21.0454603362217,-17.8483295278292,
-19.4900809580806));
#59045=CARTESIAN_POINT('Ctrl Pts',(-21.0059873754064,-17.7723079359452,
-19.4943345360339));
#59046=CARTESIAN_POINT('Ctrl Pts',(-20.967279678073,-17.697760176956,-19.4985056497431));
#59047=CARTESIAN_POINT('Ctrl Pts',(-20.9248702958461,-17.6250641047766,
-19.5026767634523));
#59048=CARTESIAN_POINT('Ctrl Pts',(-20.8789678617061,-17.5546049691487,
-19.5068478771615));
#59049=CARTESIAN_POINT('Ctrl Pts',(-20.8330808305555,-17.4841694767402,
-19.5110175912147));
#59050=CARTESIAN_POINT('Ctrl Pts',(-20.7837033262562,-17.4159698152611,
-19.5151873052678));
#59051=CARTESIAN_POINT('Ctrl Pts',(-20.7310884046656,-17.3503639914293,
-19.519357019321));
#59052=CARTESIAN_POINT('Ctrl Pts',(-20.6784753553166,-17.2847605021054,
-19.5235265849996));
#59053=CARTESIAN_POINT('Ctrl Pts',(-20.6226254062025,-17.2217510252597,
-19.5276961506783));
#59054=CARTESIAN_POINT('Ctrl Pts',(-20.5638323065115,-17.1616610013612,
-19.5318657163569));
#59055=CARTESIAN_POINT('Ctrl Pts',(-20.5029721055919,-17.0994582777943,
-19.5361818794149));
#59056=CARTESIAN_POINT('Ctrl Pts',(-20.4389583090022,-17.0403845006845,
-19.5404980424729));
#59057=CARTESIAN_POINT('Ctrl Pts',(-20.3721573781207,-16.9847581733532,
-19.5448142055309));
#59058=CARTESIAN_POINT('Ctrl Pts',(-20.3075324893086,-16.9309438750886,
-19.5489897694644));
#59059=CARTESIAN_POINT('Ctrl Pts',(-20.2402996649794,-16.8803561190116,
-19.553165333398));
#59060=CARTESIAN_POINT('Ctrl Pts',(-20.1708219663603,-16.8332403069284,
-19.5573408973316));
#59061=CARTESIAN_POINT('Ctrl Pts',(-20.0978350997288,-16.7837447772679,
-19.5617273599518));
#59062=CARTESIAN_POINT('Ctrl Pts',(-20.0223711203466,-16.738081448703,-19.566113822572));
#59063=CARTESIAN_POINT('Ctrl Pts',(-19.9448802162024,-16.6964803033426,
-19.5705002851921));
#59064=CARTESIAN_POINT('Ctrl Pts',(-19.8673893120582,-16.6548791579822,
-19.5748867478123));
#59065=CARTESIAN_POINT('Ctrl Pts',(-19.7878720403135,-16.6173403747379,
-19.5792732104325));
#59066=CARTESIAN_POINT('Ctrl Pts',(-19.706800567316,-16.5840348279103,-19.5836596730527));
#59067=CARTESIAN_POINT('Ctrl Pts',(-19.6294593229195,-16.5522617227512,
-19.587844307487));
#59068=CARTESIAN_POINT('Ctrl Pts',(-19.5504158778324,-16.5242225928466,
-19.5920289419213));
#59069=CARTESIAN_POINT('Ctrl Pts',(-19.4700654949528,-16.500101228203,-19.5962135763556));
#59070=CARTESIAN_POINT('Ctrl Pts',(-19.3898294809444,-16.4760141973502,
-19.6003922544784));
#59071=CARTESIAN_POINT('Ctrl Pts',(-19.3082906610536,-16.4558339863015,
-19.6045709326011));
#59072=CARTESIAN_POINT('Ctrl Pts',(-19.2258642779044,-16.4396963694407,
-19.6087496107238));
#59073=CARTESIAN_POINT('Ctrl Pts',(-19.1419604620519,-16.4232694975866,
-19.6130031885992));
#59074=CARTESIAN_POINT('Ctrl Pts',(-19.0571373968203,-16.4110317555328,
-19.6172567664746));
#59075=CARTESIAN_POINT('Ctrl Pts',(-18.9718493062316,-16.4030732243697,
-19.6215103443501));
#59076=CARTESIAN_POINT('Ctrl Pts',(-18.8882146908572,-16.3952689847839,
-19.6256814583605));
#59077=CARTESIAN_POINT('Ctrl Pts',(-18.8041333991978,-16.391579559832,-19.6298525723709));
#59078=CARTESIAN_POINT('Ctrl Pts',(-18.7200422944405,-16.3920380505844,
-19.6340236863813));
#59079=CARTESIAN_POINT('Ctrl Pts',(-18.6359794073137,-16.3924963874856,
-19.6381934007318));
#59080=CARTESIAN_POINT('Ctrl Pts',(-18.551907173272,-16.397099873298,-19.6423631150822));
#59081=CARTESIAN_POINT('Ctrl Pts',(-18.4682635936936,-16.4058295103502,
-19.6465328294327));
#59082=CARTESIAN_POINT('Ctrl Pts',(-18.3846229905612,-16.4145588367595,
-19.6507023954044));
#59083=CARTESIAN_POINT('Ctrl Pts',(-18.3014114690234,-16.4274139738751,
-19.6548719613761));
#59084=CARTESIAN_POINT('Ctrl Pts',(-18.2190616739277,-16.4443240798816,
-19.6590415273478));
#59085=CARTESIAN_POINT('Ctrl Pts',(-18.1338165629824,-16.4618287240758,
-19.6633576900467));
#59086=CARTESIAN_POINT('Ctrl Pts',(-18.0494954191543,-16.4836786817452,
-19.6676738527455));
#59087=CARTESIAN_POINT('Ctrl Pts',(-17.9665644117748,-16.5097382167496,
-19.6719900154444));
#59088=CARTESIAN_POINT('Ctrl Pts',(-17.8863348720819,-16.5349488655054,
-19.6761655796575));
#59089=CARTESIAN_POINT('Ctrl Pts',(-17.8074067178225,-16.5640988419262,
-19.6803411438706));
#59090=CARTESIAN_POINT('Ctrl Pts',(-17.7301828112974,-16.5970157003357,
-19.6845167080837));
#59091=CARTESIAN_POINT('Ctrl Pts',(-17.6490585105613,-16.6315951102757,
-19.6889031700254));
#59092=CARTESIAN_POINT('Ctrl Pts',(-17.5698156696774,-16.6703316765449,
-19.6932896319672));
#59093=CARTESIAN_POINT('Ctrl Pts',(-17.4928913452169,-16.7129713474315,
-19.6976760939089));
#59094=CARTESIAN_POINT('Ctrl Pts',(-17.4159670207564,-16.7556110183182,
-19.7020625558507));
#59095=CARTESIAN_POINT('Ctrl Pts',(-17.3413616647363,-16.8021534221795,
-19.7064490177924));
#59096=CARTESIAN_POINT('Ctrl Pts',(-17.2694745299275,-16.8522940330825,
-19.7108354797342));
#59097=CARTESIAN_POINT('Ctrl Pts',(-17.2373036985659,-16.8747328900772,
-19.7127985031288));
#59098=CARTESIAN_POINT('Ctrl Pts',(-17.2056206681701,-16.8979308207117,
-19.7147615265234));
#59099=CARTESIAN_POINT('Ctrl Pts',(-17.1744641548914,-16.9218650419685,
-19.7167245499181));
#59100=CARTESIAN_POINT('',(-21.2939989850553,-18.9542795868244,-19.3667098901939));
#59101=CARTESIAN_POINT('Ctrl Pts',(-21.2939989850559,-18.954279586128,-19.3667098902285));
#59102=CARTESIAN_POINT('Ctrl Pts',(-21.294073180434,-18.8709574030256,-19.3708480242597));
#59103=CARTESIAN_POINT('Ctrl Pts',(-21.2900751830219,-18.7875513930813,
-19.3749861582908));
#59104=CARTESIAN_POINT('Ctrl Pts',(-21.2820071809341,-18.7044936245096,
-19.379124292322));
#59105=CARTESIAN_POINT('Ctrl Pts',(-21.2739428344709,-18.6214734895453,
-19.3832605513581));
#59106=CARTESIAN_POINT('Ctrl Pts',(-21.2618121886764,-18.5388017480938,
-19.3873968103941));
#59107=CARTESIAN_POINT('Ctrl Pts',(-21.2456694473266,-18.4569074961523,
-19.3915330694301));
#59108=CARTESIAN_POINT('Ctrl Pts',(-21.2295289836496,-18.3750247991451,
-19.3956687448574));
#59109=CARTESIAN_POINT('Ctrl Pts',(-21.2093776397613,-18.2939198329769,
-19.3998044202847));
#59110=CARTESIAN_POINT('Ctrl Pts',(-21.1853208566141,-18.214012155975,-19.403940095712));
#59111=CARTESIAN_POINT('Ctrl Pts',(-21.1612599617833,-18.1340908214908,
-19.4080764779915));
#59112=CARTESIAN_POINT('Ctrl Pts',(-21.1332924395156,-18.0553676300856,
-19.4122128602709));
#59113=CARTESIAN_POINT('Ctrl Pts',(-21.1015733410968,-17.9782461940883,
-19.4163492425504));
#59114=CARTESIAN_POINT('Ctrl Pts',(-21.0698191717564,-17.901039487072,-19.4204901983123));
#59115=CARTESIAN_POINT('Ctrl Pts',(-21.0343053289603,-17.825438502363,-19.4246311540741));
#59116=CARTESIAN_POINT('Ctrl Pts',(-20.9952344193641,-17.7518254707406,
-19.428772109836));
#59117=CARTESIAN_POINT('Ctrl Pts',(-20.9561382227283,-17.6781647961105,
-19.4329157456612));
#59118=CARTESIAN_POINT('Ctrl Pts',(-20.9134806196083,-17.6064950352479,
-19.4370593814864));
#59119=CARTESIAN_POINT('Ctrl Pts',(-20.8675081508587,-17.5371703387972,
-19.4412030173116));
#59120=CARTESIAN_POINT('Ctrl Pts',(-20.8214607545949,-17.4677326545666,
-19.4453534065774));
#59121=CARTESIAN_POINT('Ctrl Pts',(-20.7720879921757,-17.4006480348511,
-19.4495037958431));
#59122=CARTESIAN_POINT('Ctrl Pts',(-20.7196769297237,-17.3362379102222,
-19.4536541851088));
#59123=CARTESIAN_POINT('Ctrl Pts',(-20.7018115389434,-17.3142823918094,
-19.4550689308257));
#59124=CARTESIAN_POINT('Ctrl Pts',(-20.6835934338648,-17.2926373126042,
-19.4564836765426));
#59125=CARTESIAN_POINT('Ctrl Pts',(-20.6650349200515,-17.2713143846806,
-19.4578984222595));
#59126=CARTESIAN_POINT('Ctrl Pts',(-20.6101412425931,-17.2082439287333,
-19.4620830566462));
#59127=CARTESIAN_POINT('Ctrl Pts',(-20.552052199416,-17.1477482923966,-19.4662676910329));
#59128=CARTESIAN_POINT('Ctrl Pts',(-20.4910387353975,-17.0901689436706,
-19.4704523254196));
#59129=CARTESIAN_POINT('Ctrl Pts',(-20.4301121164985,-17.0326715520257,
-19.4746310034968));
#59130=CARTESIAN_POINT('Ctrl Pts',(-20.3662696766049,-16.9780825158894,
-19.4788096815741));
#59131=CARTESIAN_POINT('Ctrl Pts',(-20.2998217436397,-16.9267093376147,
-19.4829883596513));
#59132=CARTESIAN_POINT('Ctrl Pts',(-20.2321827790971,-16.8744153319368,
-19.4872419375384));
#59133=CARTESIAN_POINT('Ctrl Pts',(-20.1618443123322,-16.8254539702931,
-19.4914955154255));
#59134=CARTESIAN_POINT('Ctrl Pts',(-20.0891719990944,-16.7801093828486,
-19.4957490933125));
#59135=CARTESIAN_POINT('Ctrl Pts',(-20.0179085806131,-16.7356438888117,
-19.4999202072829));
#59136=CARTESIAN_POINT('Ctrl Pts',(-19.9444014087305,-16.6946564386937,
-19.5040913212534));
#59137=CARTESIAN_POINT('Ctrl Pts',(-19.8690261614839,-16.6573724457448,
-19.5082624352238));
#59138=CARTESIAN_POINT('Ctrl Pts',(-19.7936762071349,-16.6201009638025,
-19.5124321495363));
#59139=CARTESIAN_POINT('Ctrl Pts',(-19.7164598343598,-16.5865306747405,
-19.5166018638488));
#59140=CARTESIAN_POINT('Ctrl Pts',(-19.6377770918967,-16.5568409305095,
-19.5207715781614));
#59141=CARTESIAN_POINT('Ctrl Pts',(-19.5590971493085,-16.527152242769,-19.5249411440973));
#59142=CARTESIAN_POINT('Ctrl Pts',(-19.4789513714909,-16.5013439869193,
-19.5291107100332));
#59143=CARTESIAN_POINT('Ctrl Pts',(-19.3977582580731,-16.4795467699389,
-19.5332802759692));
#59144=CARTESIAN_POINT('Ctrl Pts',(-19.3137104946165,-16.4569831896096,
-19.5375964387168));
#59145=CARTESIAN_POINT('Ctrl Pts',(-19.2285408859958,-16.4387180891116,
-19.5419126014644));
#59146=CARTESIAN_POINT('Ctrl Pts',(-19.1427269885612,-16.4248390932072,
-19.5462287642121));
#59147=CARTESIAN_POINT('Ctrl Pts',(-19.0597084701507,-16.4114122041898,
-19.5504043283951));
#59148=CARTESIAN_POINT('Ctrl Pts',(-18.9760874671123,-16.4020900585603,
-19.554579892578));
#59149=CARTESIAN_POINT('Ctrl Pts',(-18.8923014001436,-16.3968990887418,
-19.558755456761));
#59150=CARTESIAN_POINT('Ctrl Pts',(-18.8042834975808,-16.391445935345,-19.5631419187909));
#59151=CARTESIAN_POINT('Ctrl Pts',(-18.7160840019592,-16.3905522627805,
-19.5675283808209));
#59152=CARTESIAN_POINT('Ctrl Pts',(-18.6282074804617,-16.3941868827434,
-19.5719148428509));
#59153=CARTESIAN_POINT('Ctrl Pts',(-18.5403309589642,-16.3978215027064,
-19.5763013048809));
#59154=CARTESIAN_POINT('Ctrl Pts',(-18.4527779822414,-16.4059842855988,
-19.5806877669109));
#59155=CARTESIAN_POINT('Ctrl Pts',(-18.3660419494154,-16.4185819782338,
-19.5850742289409));
#59156=CARTESIAN_POINT('Ctrl Pts',(-18.2832980106531,-16.4305998521666,
-19.5892588006093));
#59157=CARTESIAN_POINT('Ctrl Pts',(-18.2009894838769,-16.4466981015662,
-19.5934433722777));
#59158=CARTESIAN_POINT('Ctrl Pts',(-18.1195501274547,-16.4668337371256,
-19.5976279439461));
#59159=CARTESIAN_POINT('Ctrl Pts',(-18.0344368519108,-16.4878777381211,
-19.6020012913924));
#59160=CARTESIAN_POINT('Ctrl Pts',(-17.9502735214004,-16.5133320171584,
-19.6063746388388));
#59161=CARTESIAN_POINT('Ctrl Pts',(-17.8675488473877,-16.5430868840623,
-19.6107479862852));
#59162=CARTESIAN_POINT('Ctrl Pts',(-17.7886021888952,-16.5714828535114,
-19.6149216040291));
#59163=CARTESIAN_POINT('Ctrl Pts',(-17.7109661623552,-16.6037950541263,
-19.619095221773));
#59164=CARTESIAN_POINT('Ctrl Pts',(-17.6350528481384,-16.6398764830971,
-19.623268839517));
#59165=CARTESIAN_POINT('Ctrl Pts',(-17.559191078058,-16.6759334132549,-19.6274396234296));
#59166=CARTESIAN_POINT('Ctrl Pts',(-17.4850501109929,-16.7157542909664,
-19.6316104073423));
#59167=CARTESIAN_POINT('Ctrl Pts',(-17.4130221293664,-16.7591439934879,
-19.635781191255));
#59168=CARTESIAN_POINT('Ctrl Pts',(-17.3410198802816,-16.8025181947097,
-19.6399504851235));
#59169=CARTESIAN_POINT('Ctrl Pts',(-17.2711295100132,-16.849458449815,-19.644119778992));
#59170=CARTESIAN_POINT('Ctrl Pts',(-17.2037174808643,-16.8997243334222,
-19.6482890728606));
#59171=CARTESIAN_POINT('Ctrl Pts',(-17.1939136458765,-16.9070345781162,
-19.6488954196746));
#59172=CARTESIAN_POINT('Ctrl Pts',(-17.1841621789156,-16.9144150859779,
-19.6495017664887));
#59173=CARTESIAN_POINT('Ctrl Pts',(-17.1744641548914,-16.9218650419685,
-19.6501081133027));
#59174=CARTESIAN_POINT('Ctrl Pts',(-17.1744641548914,-16.9218650419685,
-18.8501886385061));
#59175=CARTESIAN_POINT('Ctrl Pts',(-17.1079119429244,-16.9729899978358,
-18.8543616936919));
#59176=CARTESIAN_POINT('Ctrl Pts',(-17.0438080821223,-17.0274434278499,
-18.8585347488777));
#59177=CARTESIAN_POINT('Ctrl Pts',(-16.9824992587632,-17.0849581811199,
-18.8627078040634));
#59178=CARTESIAN_POINT('Ctrl Pts',(-16.9212252296614,-17.1424402933604,
-18.8668784909383));
#59179=CARTESIAN_POINT('Ctrl Pts',(-16.8627434233976,-17.2029799654239,
-18.8710491778132));
#59180=CARTESIAN_POINT('Ctrl Pts',(-16.8073667378616,-17.2662704032906,
-18.875219864688));
#59181=CARTESIAN_POINT('Ctrl Pts',(-16.7520048680834,-17.3295439081143,
-18.8793894357163));
#59182=CARTESIAN_POINT('Ctrl Pts',(-16.6997467716427,-17.3955663708758,
-18.8835590067445));
#59183=CARTESIAN_POINT('Ctrl Pts',(-16.6508668661375,-17.4639958512813,
-18.8877285777728));
#59184=CARTESIAN_POINT('Ctrl Pts',(-16.601985375499,-17.5324275507959,-18.8918982840166));
#59185=CARTESIAN_POINT('Ctrl Pts',(-16.5564825596719,-17.6032660478446,
-18.8960679902605));
#59186=CARTESIAN_POINT('Ctrl Pts',(-16.5145902773873,-17.6761393167072,
-18.9002376965043));
#59187=CARTESIAN_POINT('Ctrl Pts',(-16.4726552587905,-17.7490869270619,
-18.9044116564641));
#59188=CARTESIAN_POINT('Ctrl Pts',(-16.4343383603789,-17.8240730555622,
-18.9085856164239));
#59189=CARTESIAN_POINT('Ctrl Pts',(-16.3998258519895,-17.9007003059263,
-18.9127595763837));
#59190=CARTESIAN_POINT('Ctrl Pts',(-16.3652960238365,-17.9773660109238,
-18.9169356310043));
#59191=CARTESIAN_POINT('Ctrl Pts',(-16.3345745566648,-18.0556740495226,
-18.9211116856249));
#59192=CARTESIAN_POINT('Ctrl Pts',(-16.3077989187118,-18.1352085252919,
-18.9252877402455));
#59193=CARTESIAN_POINT('Ctrl Pts',(-16.2809754720839,-18.2148850121648,
-18.9294712513322));
#59194=CARTESIAN_POINT('Ctrl Pts',(-16.2581120567994,-18.2957918679272,
-18.9336547624189));
#59195=CARTESIAN_POINT('Ctrl Pts',(-16.2392957334692,-18.3774996757589,
-18.9378382735057));
#59196=CARTESIAN_POINT('Ctrl Pts',(-16.2222689257246,-18.4514367096189,
-18.9416239141817));
#59197=CARTESIAN_POINT('Ctrl Pts',(-16.2085553942316,-18.5260292086691,
-18.9454095548577));
#59198=CARTESIAN_POINT('Ctrl Pts',(-16.1981829862585,-18.6009557395151,
-18.9491951955337));
#59199=CARTESIAN_POINT('Ctrl Pts',(-16.1867173615959,-18.6837792730849,
-18.9533798299225));
#59200=CARTESIAN_POINT('Ctrl Pts',(-16.1792923755172,-18.7673192548711,
-18.9575644643113));
#59201=CARTESIAN_POINT('Ctrl Pts',(-16.1759873564286,-18.8511470608817,
-18.9617490987001));
#59202=CARTESIAN_POINT('Ctrl Pts',(-16.1726870416255,-18.9348555483864,
-18.9659277767798));
#59203=CARTESIAN_POINT('Ctrl Pts',(-16.173495063509,-19.0188505906137,-18.9701064548595));
#59204=CARTESIAN_POINT('Ctrl Pts',(-16.1784392678898,-19.1026961993429,
-18.9742851329392));
#59205=CARTESIAN_POINT('Ctrl Pts',(-16.1834720935872,-19.1880446804577,
-18.9785387108257));
#59206=CARTESIAN_POINT('Ctrl Pts',(-16.1927909085455,-19.2732378406054,
-18.9827922887122));
#59207=CARTESIAN_POINT('Ctrl Pts',(-16.2063695825694,-19.3578133473403,
-18.9870458665987));
#59208=CARTESIAN_POINT('Ctrl Pts',(-16.219685007484,-19.4407491927378,-18.9912169805725));
#59209=CARTESIAN_POINT('Ctrl Pts',(-16.2370965177703,-19.523090644708,-18.9953880945462));
#59210=CARTESIAN_POINT('Ctrl Pts',(-16.2585271389983,-19.6044064028226,
-18.99955920852));
#59211=CARTESIAN_POINT('Ctrl Pts',(-16.2799505689745,-19.6856948746498,
-19.0037289228362));
#59212=CARTESIAN_POINT('Ctrl Pts',(-16.3053903143092,-19.7659578916983,
-19.0078986371525));
#59213=CARTESIAN_POINT('Ctrl Pts',(-16.3347186663492,-19.8447760536634,
-19.0120683514687));
#59214=CARTESIAN_POINT('Ctrl Pts',(-16.3640459747608,-19.9235914109408,
-19.0162379174086));
#59215=CARTESIAN_POINT('Ctrl Pts',(-16.3972614535252,-20.0009615845049,
-19.0204074833486));
#59216=CARTESIAN_POINT('Ctrl Pts',(-16.4341885271964,-20.0764852998421,
-19.0245770492885));
#59217=CARTESIAN_POINT('Ctrl Pts',(-16.4724139113051,-20.154664336009,-19.0288932120324));
#59218=CARTESIAN_POINT('Ctrl Pts',(-16.5146165141599,-20.2308641813284,
-19.0332093747763));
#59219=CARTESIAN_POINT('Ctrl Pts',(-16.5605485527335,-20.3046672933043,
-19.0375255375201));
#59220=CARTESIAN_POINT('Ctrl Pts',(-16.6049843598883,-20.37606627652,-19.0417011017079));
#59221=CARTESIAN_POINT('Ctrl Pts',(-16.6529100541809,-20.4452219153925,
-19.0458766658956));
#59222=CARTESIAN_POINT('Ctrl Pts',(-16.7040581042265,-20.5117871328432,
-19.0500522300833));
#59223=CARTESIAN_POINT('Ctrl Pts',(-16.7577895208536,-20.5817144014007,
-19.0544386921052));
#59224=CARTESIAN_POINT('Ctrl Pts',(-16.8150769912941,-20.6487822429873,
-19.0588251541272));
#59225=CARTESIAN_POINT('Ctrl Pts',(-16.8755654265139,-20.712630834693,-19.0632116161492));
#59226=CARTESIAN_POINT('Ctrl Pts',(-16.9360538617338,-20.7764794263986,
-19.0675980781712));
#59227=CARTESIAN_POINT('Ctrl Pts',(-16.9997427890404,-20.8371084232607,
-19.0719845401931));
#59228=CARTESIAN_POINT('Ctrl Pts',(-17.066237677054,-20.8942072068041,-19.0763710022151));
#59229=CARTESIAN_POINT('Ctrl Pts',(-17.1296730365257,-20.9486787905254,
-19.0805556366056));
#59230=CARTESIAN_POINT('Ctrl Pts',(-17.1958979365974,-21.0001406364728,
-19.0847402709961));
#59231=CARTESIAN_POINT('Ctrl Pts',(-17.2645949112844,-21.0482940359732,
-19.0889249053866));
#59232=CARTESIAN_POINT('Ctrl Pts',(-17.3331941043301,-21.096378895069,-19.0931035834679));
#59233=CARTESIAN_POINT('Ctrl Pts',(-17.4042580092783,-21.1411643998052,
-19.0972822615492));
#59234=CARTESIAN_POINT('Ctrl Pts',(-17.4774351014414,-21.1823911441069,
-19.1014609396306));
#59235=CARTESIAN_POINT('Ctrl Pts',(-17.551923840448,-21.2243568482037,-19.1057145175167));
#59236=CARTESIAN_POINT('Ctrl Pts',(-17.6286019037977,-21.2626346413132,
-19.1099680954027));
#59237=CARTESIAN_POINT('Ctrl Pts',(-17.7070663992904,-21.2969962430106,
-19.1142216732888));
#59238=CARTESIAN_POINT('Ctrl Pts',(-17.7840097073652,-21.3306916779808,
-19.1183927872641));
#59239=CARTESIAN_POINT('Ctrl Pts',(-17.8626703579571,-21.3606212194832,
-19.1225639012393));
#59240=CARTESIAN_POINT('Ctrl Pts',(-17.9426440308619,-21.3866161360899,
-19.1267350152145));
#59241=CARTESIAN_POINT('Ctrl Pts',(-18.0225908678278,-21.4126023298512,
-19.1309047295321));
#59242=CARTESIAN_POINT('Ctrl Pts',(-18.103849414936,-21.4346563787677,-19.1350744438498));
#59243=CARTESIAN_POINT('Ctrl Pts',(-18.1859978966301,-21.4526586521759,
-19.1392441581674));
#59244=CARTESIAN_POINT('Ctrl Pts',(-18.2681434551281,-21.4706602849858,
-19.1434137241086));
#59245=CARTESIAN_POINT('Ctrl Pts',(-18.3511784356968,-21.4846103313097,
-19.1475832900499));
#59246=CARTESIAN_POINT('Ctrl Pts',(-18.4346698530335,-21.4944400608701,
-19.1517528559912));
#59247=CARTESIAN_POINT('Ctrl Pts',(-18.5210967257278,-21.5046153916099,
-19.1560690187333));
#59248=CARTESIAN_POINT('Ctrl Pts',(-18.608012205207,-21.5103752123295,-19.1603851814754));
#59249=CARTESIAN_POINT('Ctrl Pts',(-18.6949310840572,-21.5117018615079,
-19.1647013442175));
#59250=CARTESIAN_POINT('Ctrl Pts',(-18.7790185894518,-21.5129852952271,
-19.1688769084064));
#59251=CARTESIAN_POINT('Ctrl Pts',(-18.8631088069887,-21.5101200064032,
-19.1730524725952));
#59252=CARTESIAN_POINT('Ctrl Pts',(-18.9467650901062,-21.5031430803528,
-19.1772280367841));
#59253=CARTESIAN_POINT('Ctrl Pts',(-19.0346466533943,-21.4958137663384,
-19.1816144988028));
#59254=CARTESIAN_POINT('Ctrl Pts',(-19.1220487155994,-21.483946620245,-19.1860009608216));
#59255=CARTESIAN_POINT('Ctrl Pts',(-19.2084765196392,-21.4676454504383,
-19.1903874228403));
#59256=CARTESIAN_POINT('Ctrl Pts',(-19.2949043236791,-21.4513442806317,
-19.1947738848591));
#59257=CARTESIAN_POINT('Ctrl Pts',(-19.380357323635,-21.43060929785,-19.1991603468779));
#59258=CARTESIAN_POINT('Ctrl Pts',(-19.4643607861739,-21.4056041086572,
-19.2035468088966));
#59259=CARTESIAN_POINT('Ctrl Pts',(-19.5444991251693,-21.3817494451991,
-19.2077314433108));
#59260=CARTESIAN_POINT('Ctrl Pts',(-19.6236166763929,-21.3539201055357,
-19.211916077725));
#59261=CARTESIAN_POINT('Ctrl Pts',(-19.7012904348026,-21.3222213429846,
-19.2161007121391));
#59262=CARTESIAN_POINT('Ctrl Pts',(-19.778853634233,-21.2905676996977,-19.2202793902443));
#59263=CARTESIAN_POINT('Ctrl Pts',(-19.8549767005595,-21.2550557457739,
-19.2244580683494));
#59264=CARTESIAN_POINT('Ctrl Pts',(-19.9292512406756,-21.215840646261,-19.2286367464546));
#59265=CARTESIAN_POINT('Ctrl Pts',(-20.0048570980657,-21.1759226445248,
-19.2328903243347));
#59266=CARTESIAN_POINT('Ctrl Pts',(-20.0785470456786,-21.1321675712325,
-19.2371439022148));
#59267=CARTESIAN_POINT('Ctrl Pts',(-20.1499110579027,-21.0847906311002,
-19.241397480095));
#59268=CARTESIAN_POINT('Ctrl Pts',(-20.2198915399371,-21.038332185107,-19.2455685940941));
#59269=CARTESIAN_POINT('Ctrl Pts',(-20.2876350664325,-20.9883913190918,
-19.2497397080933));
#59270=CARTESIAN_POINT('Ctrl Pts',(-20.3527809100999,-20.935216671243,-19.2539108220924));
#59271=CARTESIAN_POINT('Ctrl Pts',(-20.4179048934498,-20.8820598666613,
-19.2580805364339));
#59272=CARTESIAN_POINT('Ctrl Pts',(-20.480432569049,-20.8256717259784,-19.2622502507755));
#59273=CARTESIAN_POINT('Ctrl Pts',(-20.5400350473299,-20.766342141884,-19.266419965117));
#59274=CARTESIAN_POINT('Ctrl Pts',(-20.5996354046978,-20.7070146689917,
-19.2705895310821));
#59275=CARTESIAN_POINT('Ctrl Pts',(-20.6563104462705,-20.6447462859464,
-19.2747590970472));
#59276=CARTESIAN_POINT('Ctrl Pts',(-20.7097680140269,-20.5798638624738,
-19.2789286630123));
#59277=CARTESIAN_POINT('Ctrl Pts',(-20.7651050833169,-20.5127002537634,
-19.2832448257261));
#59278=CARTESIAN_POINT('Ctrl Pts',(-20.8169938810791,-20.4427357722886,
-19.2875609884399));
#59279=CARTESIAN_POINT('Ctrl Pts',(-20.8651569232062,-20.3703688408415,
-19.2918771511538));
#59280=CARTESIAN_POINT('Ctrl Pts',(-20.9117510598039,-20.3003592538204,
-19.2960527153661));
#59281=CARTESIAN_POINT('Ctrl Pts',(-20.9548582452865,-20.2281017614681,
-19.3002282795785));
#59282=CARTESIAN_POINT('Ctrl Pts',(-20.9942733140313,-20.1539835880236,
-19.3044038437909));
#59283=CARTESIAN_POINT('Ctrl Pts',(-21.0356791435396,-20.0761218830757,
-19.3087903057554));
#59284=CARTESIAN_POINT('Ctrl Pts',(-21.0730098296578,-19.9962071202703,
-19.3131767677199));
#59285=CARTESIAN_POINT('Ctrl Pts',(-21.1060848561741,-19.9147115014943,
-19.3175632296844));
#59286=CARTESIAN_POINT('Ctrl Pts',(-21.1391598826905,-19.8332158827183,
-19.321949691649));
#59287=CARTESIAN_POINT('Ctrl Pts',(-21.1679791313071,-19.7501399810715,
-19.3263361536135));
#59288=CARTESIAN_POINT('Ctrl Pts',(-21.1924232051046,-19.6659715292665,
-19.330722615578));
#59289=CARTESIAN_POINT('Ctrl Pts',(-21.2214742546437,-19.56593984538,-19.3359357942359));
#59290=CARTESIAN_POINT('Ctrl Pts',(-21.2444357643464,-19.4640653478474,
-19.3411489728938));
#59291=CARTESIAN_POINT('Ctrl Pts',(-21.261115150052,-19.3610098023001,-19.3463621515516));
#59292=CARTESIAN_POINT('Ctrl Pts',(-21.277528721009,-19.2595966244285,-19.3514922492257));
#59293=CARTESIAN_POINT('Ctrl Pts',(-21.2878587862943,-19.1570396545895,
-19.3566223468997));
#59294=CARTESIAN_POINT('Ctrl Pts',(-21.2919675308073,-19.0539907414198,
-19.3617524445737));
#59295=CARTESIAN_POINT('Ctrl Pts',(-21.2932910194155,-19.020797131491,-19.3634049264471));
#59296=CARTESIAN_POINT('Ctrl Pts',(-21.2939693565913,-18.9875526505269,
-19.3650574083205));
#59297=CARTESIAN_POINT('Ctrl Pts',(-21.2939989850553,-18.9542795868244,
-19.3667098901939));
#59298=CARTESIAN_POINT('Origin',(-18.734,-18.952,1.76670989022851));
#59299=CARTESIAN_POINT('',(-17.1744641548914,-16.9218650419685,-18.0500683176023));
#59300=CARTESIAN_POINT('',(-17.1744641548915,-16.9218650419685,-18.1167065540548));
#59301=CARTESIAN_POINT('',(-17.1744641548914,-16.9218650419685,1.76670989022851));
#59302=CARTESIAN_POINT('',(-21.2936055493641,-18.9516176052657,-18.6332901348852));
#59303=CARTESIAN_POINT('Ctrl Pts',(-17.1744641548915,-16.9218650419685,
-18.1167065540548));
#59304=CARTESIAN_POINT('Ctrl Pts',(-17.1077794165571,-16.9730918036883,
-18.1208760334781));
#59305=CARTESIAN_POINT('Ctrl Pts',(-17.0436129585211,-17.027614071718,-18.1250455129013));
#59306=CARTESIAN_POINT('Ctrl Pts',(-16.9822980504549,-17.0851469581245,
-18.1292149923245));
#59307=CARTESIAN_POINT('Ctrl Pts',(-16.920972396523,-17.1426899275709,-18.1333852024781));
#59308=CARTESIAN_POINT('Ctrl Pts',(-16.8624996194374,-17.2032442473846,
-18.1375554126317));
#59309=CARTESIAN_POINT('Ctrl Pts',(-16.8071766738075,-17.2664876536672,
-18.1417256227852));
#59310=CARTESIAN_POINT('Ctrl Pts',(-16.7517926209873,-17.3298009157179,
-18.1459004391618));
#59311=CARTESIAN_POINT('Ctrl Pts',(-16.6995656464103,-17.3958088452489,
-18.1500752555384));
#59312=CARTESIAN_POINT('Ctrl Pts',(-16.650752512836,-17.4641559533254,-18.154250071915));
#59313=CARTESIAN_POINT('Ctrl Pts',(-16.6019086309308,-17.532546114559,-18.1584275180887));
#59314=CARTESIAN_POINT('Ctrl Pts',(-16.5564831185187,-17.603278000295,-18.1626049642624));
#59315=CARTESIAN_POINT('Ctrl Pts',(-16.5146881815939,-17.6759690236193,
-18.166782410436));
#59316=CARTESIAN_POINT('Ctrl Pts',(-16.472824736,-17.7487791993012,-18.1709667041204));
#59317=CARTESIAN_POINT('Ctrl Pts',(-16.434603952541,-17.8235545130221,-18.1751509978048));
#59318=CARTESIAN_POINT('Ctrl Pts',(-16.400190878549,-17.8998902221573,-18.1793352914892));
#59319=CARTESIAN_POINT('Ctrl Pts',(-16.3854130795555,-17.9326706057374,
-18.1811321275118));
#59320=CARTESIAN_POINT('Ctrl Pts',(-16.3713368223245,-17.9657385181925,
-18.1829289635344));
#59321=CARTESIAN_POINT('Ctrl Pts',(-16.3579723492966,-17.9990610706384,
-18.184725799557));
#59322=CARTESIAN_POINT('Ctrl Pts',(-16.3268479546497,-18.0766656473996,
-18.1889104339505));
#59323=CARTESIAN_POINT('Ctrl Pts',(-16.2994716572955,-18.1559410996701,
-18.193095068344));
#59324=CARTESIAN_POINT('Ctrl Pts',(-16.2760239311543,-18.236490639487,-18.1972797027375));
#59325=CARTESIAN_POINT('Ctrl Pts',(-16.2526095799489,-18.3169255270041,
-18.2014583808218));
#59326=CARTESIAN_POINT('Ctrl Pts',(-16.2331128202904,-18.398630461953,-18.2056370589062));
#59327=CARTESIAN_POINT('Ctrl Pts',(-16.217665944864,-18.4811890793931,-18.2098157369906));
#59328=CARTESIAN_POINT('Ctrl Pts',(-16.201942195299,-18.565227500706,-18.2140693148759));
#59329=CARTESIAN_POINT('Ctrl Pts',(-16.1904151258529,-18.6501500625611,
-18.2183228927612));
#59330=CARTESIAN_POINT('Ctrl Pts',(-16.1831710111198,-18.7355018025745,
-18.2225764706466));
#59331=CARTESIAN_POINT('Ctrl Pts',(-16.1760673376856,-18.8191988325684,
-18.226747584625));
#59332=CARTESIAN_POINT('Ctrl Pts',(-16.1730820747445,-18.9033080688141,
-18.2309186986033));
#59333=CARTESIAN_POINT('Ctrl Pts',(-16.1742446642318,-18.9873923862777,
-18.2350898125817));
#59334=CARTESIAN_POINT('Ctrl Pts',(-16.1754068636011,-19.0714484884366,
-18.2392595269025));
#59335=CARTESIAN_POINT('Ctrl Pts',(-16.180714144804,-19.1554792288139,-18.2434292412234));
#59336=CARTESIAN_POINT('Ctrl Pts',(-16.1901438433303,-19.2390467804617,
-18.2475989555442));
#59337=CARTESIAN_POINT('Ctrl Pts',(-16.1995732063073,-19.3226113584171,
-18.2517685214886));
#59338=CARTESIAN_POINT('Ctrl Pts',(-16.2131246425146,-19.4057123233778,
-18.2559380874331));
#59339=CARTESIAN_POINT('Ctrl Pts',(-16.2307236899664,-19.4879176388445,
-18.2601076533776));
#59340=CARTESIAN_POINT('Ctrl Pts',(-16.2489414982119,-19.573013191773,-18.264423816116));
#59341=CARTESIAN_POINT('Ctrl Pts',(-16.2714967310845,-19.6571484255569,
-18.2687399788544));
#59342=CARTESIAN_POINT('Ctrl Pts',(-16.2982497538329,-19.7398583237466,
-18.2730561415928));
#59343=CARTESIAN_POINT('Ctrl Pts',(-16.3241312996849,-19.8198739557201,
-18.2772317057849));
#59344=CARTESIAN_POINT('Ctrl Pts',(-16.3539411382348,-19.8985552629114,
-18.281407269977));
#59345=CARTESIAN_POINT('Ctrl Pts',(-16.3875034565753,-19.9755008410821,
-18.2855828341691));
#59346=CARTESIAN_POINT('Ctrl Pts',(-16.4227609278168,-20.0563327574591,
-18.2899692961806));
#59347=CARTESIAN_POINT('Ctrl Pts',(-16.4621596558346,-20.1352484709665,
-18.2943557581922));
#59348=CARTESIAN_POINT('Ctrl Pts',(-16.5054419382129,-20.2118130675793,
-18.2987422202037));
#59349=CARTESIAN_POINT('Ctrl Pts',(-16.5487242205912,-20.2883776641921,
-18.3031286822153));
#59350=CARTESIAN_POINT('Ctrl Pts',(-16.5958896819153,-20.362590695021,-18.3075151442268));
#59351=CARTESIAN_POINT('Ctrl Pts',(-16.6466304638568,-20.4340554711552,
-18.3119016062384));
#59352=CARTESIAN_POINT('Ctrl Pts',(-16.6950365872103,-20.5022320470105,
-18.3160862406309));
#59353=CARTESIAN_POINT('Ctrl Pts',(-16.7468764264203,-20.5681614794156,
-18.3202708750235));
#59354=CARTESIAN_POINT('Ctrl Pts',(-16.8019140327134,-20.6314772445658,
-18.324455509416));
#59355=CARTESIAN_POINT('Ctrl Pts',(-16.8568732997864,-20.6947028875613,
-18.3286341874995));
#59356=CARTESIAN_POINT('Ctrl Pts',(-16.9150209937603,-20.755321908626,-18.3328128655829));
#59357=CARTESIAN_POINT('Ctrl Pts',(-16.976078625133,-20.8129977001022,-18.3369915436664));
#59358=CARTESIAN_POINT('Ctrl Pts',(-17.0382306706759,-20.8717072886985,
-18.3412451215519));
#59359=CARTESIAN_POINT('Ctrl Pts',(-17.1033977218493,-20.9273667019601,
-18.3454986994375));
#59360=CARTESIAN_POINT('Ctrl Pts',(-17.1712439260889,-20.9796571340969,
-18.349752277323));
#59361=CARTESIAN_POINT('Ctrl Pts',(-17.2377747992587,-21.0309338141629,
-18.3539233913005));
#59362=CARTESIAN_POINT('Ctrl Pts',(-17.3068814901404,-21.0789706821841,
-18.358094505278));
#59363=CARTESIAN_POINT('Ctrl Pts',(-17.3782123821184,-21.1235063746623,
-18.3622656192554));
#59364=CARTESIAN_POINT('Ctrl Pts',(-17.4495193383267,-21.1680271227587,
-18.3664353335753));
#59365=CARTESIAN_POINT('Ctrl Pts',(-17.5230486234685,-21.2090487851565,
-18.3706050478952));
#59366=CARTESIAN_POINT('Ctrl Pts',(-17.5984198264987,-21.2463534316994,
-18.3747747622151));
#59367=CARTESIAN_POINT('Ctrl Pts',(-17.6737883474982,-21.2836567507829,
-18.3789443281586));
#59368=CARTESIAN_POINT('Ctrl Pts',(-17.750998243395,-21.3172431136927,-18.3831138941022));
#59369=CARTESIAN_POINT('Ctrl Pts',(-17.8296459350042,-21.346941278012,-18.3872834600458));
#59370=CARTESIAN_POINT('Ctrl Pts',(-17.9110587824485,-21.3776835931598,
-18.3915996227853));
#59371=CARTESIAN_POINT('Ctrl Pts',(-17.994011919152,-21.4042590180671,-18.3959157855248));
#59372=CARTESIAN_POINT('Ctrl Pts',(-18.0780387582278,-21.4265332588779,
-18.4002319482643));
#59373=CARTESIAN_POINT('Ctrl Pts',(-18.1593284318388,-21.4480819186317,
-18.4044075124555));
#59374=CARTESIAN_POINT('Ctrl Pts',(-18.2416224598005,-21.4656052611969,
-18.4085830766467));
#59375=CARTESIAN_POINT('Ctrl Pts',(-18.3244881604797,-21.4790338449045,
-18.4127586408379));
#59376=CARTESIAN_POINT('Ctrl Pts',(-18.4115392107375,-21.4931406744569,
-18.4171451028516));
#59377=CARTESIAN_POINT('Ctrl Pts',(-18.4992206213759,-21.5027281581545,
-18.4215315648652));
#59378=CARTESIAN_POINT('Ctrl Pts',(-18.5870272090958,-21.5077775722339,
-18.4259180268789));
#59379=CARTESIAN_POINT('Ctrl Pts',(-18.6748337968157,-21.5128269863133,
-18.4303044888925));
#59380=CARTESIAN_POINT('Ctrl Pts',(-18.7627649809675,-21.5133384034635,
-18.4346909509062));
#59381=CARTESIAN_POINT('Ctrl Pts',(-18.8503205710794,-21.5093559636358,
-18.4390774129198));
#59382=CARTESIAN_POINT('Ctrl Pts',(-18.9338475986689,-21.5055567617696,
-18.4432620473123));
#59383=CARTESIAN_POINT('Ctrl Pts',(-19.0173437395028,-21.4976540121366,
-18.4474466817047));
#59384=CARTESIAN_POINT('Ctrl Pts',(-19.100373090469,-21.4856477179316,-18.4516313160972));
#59385=CARTESIAN_POINT('Ctrl Pts',(-19.1832842594309,-21.4736585132005,
-18.4558099941805));
#59386=CARTESIAN_POINT('Ctrl Pts',(-19.2657295068645,-21.4575774310127,
-18.4599886722639));
#59387=CARTESIAN_POINT('Ctrl Pts',(-19.3472750579131,-21.437456437627,-18.4641673503472));
#59388=CARTESIAN_POINT('Ctrl Pts',(-19.4302822543734,-21.4169747898919,
-18.4684209282328));
#59389=CARTESIAN_POINT('Ctrl Pts',(-19.5123567014418,-21.3923069974992,
-18.4726745061184));
#59390=CARTESIAN_POINT('Ctrl Pts',(-19.5930485432779,-21.3635628957778,
-18.476928084004));
#59391=CARTESIAN_POINT('Ctrl Pts',(-19.6721760162886,-21.3353760545629,
-18.4810991979813));
#59392=CARTESIAN_POINT('Ctrl Pts',(-19.7499735613546,-21.3032697094725,
-18.4852703119587));
#59393=CARTESIAN_POINT('Ctrl Pts',(-19.8260310897304,-21.2673980433313,
-18.489441425936));
#59394=CARTESIAN_POINT('Ctrl Pts',(-19.9020630962677,-21.2315384142742,
-18.4936111402558));
#59395=CARTESIAN_POINT('Ctrl Pts',(-19.976355829977,-21.1919161695522,-18.4977808545756));
#59396=CARTESIAN_POINT('Ctrl Pts',(-20.0485201368015,-21.1487332131925,
-18.5019505688953));
#59397=CARTESIAN_POINT('Ctrl Pts',(-20.1206818757105,-21.1055517934677,
-18.5061201348388));
#59398=CARTESIAN_POINT('Ctrl Pts',(-20.1907149440062,-21.058810150979,-18.5102897007822));
#59399=CARTESIAN_POINT('Ctrl Pts',(-20.2582569041576,-21.0087549416807,
-18.5144592667256));
#59400=CARTESIAN_POINT('Ctrl Pts',(-20.3281735563277,-20.9569398529571,
-18.5187754294653));
#59401=CARTESIAN_POINT('Ctrl Pts',(-20.3954202425924,-20.9015741660664,
-18.5230915922049));
#59402=CARTESIAN_POINT('Ctrl Pts',(-20.4596314884387,-20.8429775160242,
-18.5274077549446));
#59403=CARTESIAN_POINT('Ctrl Pts',(-20.521751059686,-20.7862896457115,-18.5315833191356));
#59404=CARTESIAN_POINT('Ctrl Pts',(-20.5810296141591,-20.7265784444844,
-18.5357588833267));
#59405=CARTESIAN_POINT('Ctrl Pts',(-20.6371745600423,-20.6641701416646,
-18.5399344475178));
#59406=CARTESIAN_POINT('Ctrl Pts',(-20.6961552536973,-20.5986097438009,
-18.5443209095317));
#59407=CARTESIAN_POINT('Ctrl Pts',(-20.7516770948085,-20.5300730764181,
-18.5487073715456));
#59408=CARTESIAN_POINT('Ctrl Pts',(-20.8034508935154,-20.458974783906,-18.5530938335595));
#59409=CARTESIAN_POINT('Ctrl Pts',(-20.8552246922222,-20.3878764913939,
-18.5574802955735));
#59410=CARTESIAN_POINT('Ctrl Pts',(-20.9032501953501,-20.3142171013321,
-18.5618667575874));
#59411=CARTESIAN_POINT('Ctrl Pts',(-20.9472937739973,-20.238441086869,-18.5662532196013));
#59412=CARTESIAN_POINT('Ctrl Pts',(-20.9909726387703,-20.1632925546555,
-18.5706033584189));
#59413=CARTESIAN_POINT('Ctrl Pts',(-21.0308877830082,-20.0858014915382,
-18.5749534972364));
#59414=CARTESIAN_POINT('Ctrl Pts',(-21.066791372662,-20.0063644586356,-18.579303636054));
#59415=CARTESIAN_POINT('Ctrl Pts',(-21.1039225287105,-19.9242114234328,
-18.5838025088638));
#59416=CARTESIAN_POINT('Ctrl Pts',(-21.1367625751618,-19.839977276334,-18.5883013816736));
#59417=CARTESIAN_POINT('Ctrl Pts',(-21.1650869626509,-19.7541322709059,
-18.5928002544834));
#59418=CARTESIAN_POINT('Ctrl Pts',(-21.1923645588308,-19.6714598603191,
-18.5971328613515));
#59419=CARTESIAN_POINT('Ctrl Pts',(-21.2154541944231,-19.5872939815202,
-18.6014654682196));
#59420=CARTESIAN_POINT('Ctrl Pts',(-21.2342029378176,-19.5020775124729,
-18.6057980750877));
#59421=CARTESIAN_POINT('Ctrl Pts',(-21.252927481766,-19.4169710343355,-18.6101250897577));
#59422=CARTESIAN_POINT('Ctrl Pts',(-21.267322189726,-19.330817060707,-18.6144521044277));
#59423=CARTESIAN_POINT('Ctrl Pts',(-21.2772839154191,-19.2440734934402,
-18.6187791190978));
#59424=CARTESIAN_POINT('Ctrl Pts',(-21.2872318317731,-19.1574501735453,
-18.6231001354886));
#59425=CARTESIAN_POINT('Ctrl Pts',(-21.2927589555484,-19.0702392928319,
-18.6274211518793));
#59426=CARTESIAN_POINT('Ctrl Pts',(-21.2938134141943,-18.9829076772209,
-18.6317421682701));
#59427=CARTESIAN_POINT('Ctrl Pts',(-21.2939393290371,-18.9724792486627,
-18.6322581487706));
#59428=CARTESIAN_POINT('Ctrl Pts',(-21.2940015277989,-18.9620491070299,
-18.632774129271));
#59429=CARTESIAN_POINT('Ctrl Pts',(-21.2939999715072,-18.9516180532908,
-18.6332901097715));
#59430=CARTESIAN_POINT('Ctrl Pts',(-21.2898370902887,-18.9516133246636,
-18.6332903748308));
#59431=CARTESIAN_POINT('Ctrl Pts',(-21.2903731169848,-18.5470182197254,
-18.6533365919814));
#59432=CARTESIAN_POINT('Ctrl Pts',(-21.0089153450218,-17.2875283998103,
-18.7157747446925));
#59433=CARTESIAN_POINT('Ctrl Pts',(-19.2309396615754,-16.0736326248611,
-18.8102032524889));
#59434=CARTESIAN_POINT('Ctrl Pts',(-17.6886694270821,-16.5353972584879,
-18.8845855431345));
#59435=CARTESIAN_POINT('Ctrl Pts',(-17.1746506085039,-16.9221163620955,
-18.9165758982197));
#59436=CARTESIAN_POINT('',(-21.2939999971965,-18.9518801919504,-18.5667098901964));
#59437=CARTESIAN_POINT('Ctrl Pts',(-21.2939999971965,-18.9518801913084,
-18.5667098902285));
#59438=CARTESIAN_POINT('Ctrl Pts',(-21.2939996986147,-18.945500276023,-18.5670291853155));
#59439=CARTESIAN_POINT('Ctrl Pts',(-21.2939755504833,-18.939120426077,-18.5673484804024));
#59440=CARTESIAN_POINT('Ctrl Pts',(-21.2939275539577,-18.9327407557766,
-18.5676677754894));
#59441=CARTESIAN_POINT('Ctrl Pts',(-21.2932985185608,-18.84912973624,-18.5718524098819));
#59442=CARTESIAN_POINT('Ctrl Pts',(-21.2885677156651,-18.7653939703417,
-18.5760370442745));
#59443=CARTESIAN_POINT('Ctrl Pts',(-21.2797186185528,-18.6819690477864,
-18.580221678667));
#59444=CARTESIAN_POINT('Ctrl Pts',(-21.2708821170351,-18.5986628702825,
-18.5844003567505));
#59445=CARTESIAN_POINT('Ctrl Pts',(-21.2579390129528,-18.5156671108363,
-18.5885790348339));
#59446=CARTESIAN_POINT('Ctrl Pts',(-21.2409247859828,-18.4334172029223,
-18.5927577129174));
#59447=CARTESIAN_POINT('Ctrl Pts',(-21.2236055912197,-18.3496930245084,
-18.5970112908029));
#59448=CARTESIAN_POINT('Ctrl Pts',(-21.2020678918843,-18.2667421815314,
-18.6012648686885));
#59449=CARTESIAN_POINT('Ctrl Pts',(-21.1764043852929,-18.1850183713399,
-18.605518446574));
#59450=CARTESIAN_POINT('Ctrl Pts',(-21.1512384158586,-18.1048789366916,
-18.6096895605515));
#59451=CARTESIAN_POINT('Ctrl Pts',(-21.1221053294157,-18.02591984166,-18.613860674529));
#59452=CARTESIAN_POINT('Ctrl Pts',(-21.0891436468891,-17.9485567268061,
-18.6180317885064));
#59453=CARTESIAN_POINT('Ctrl Pts',(-21.0561930249733,-17.8712195718925,
-18.6222015028263));
#59454=CARTESIAN_POINT('Ctrl Pts',(-21.0194165386218,-17.7954777564205,
-18.6263712171462));
#59455=CARTESIAN_POINT('Ctrl Pts',(-20.9790011895035,-17.721727810959,-18.6305409314661));
#59456=CARTESIAN_POINT('Ctrl Pts',(-20.9385872785368,-17.6479804898368,
-18.6347104974097));
#59457=CARTESIAN_POINT('Ctrl Pts',(-20.8945349840831,-17.5762253008168,
-18.6388800633532));
#59458=CARTESIAN_POINT('Ctrl Pts',(-20.8470770406693,-17.5068337741989,
-18.6430496292968));
#59459=CARTESIAN_POINT('Ctrl Pts',(-20.7979505344986,-17.4350025270909,
-18.6473657920363));
#59460=CARTESIAN_POINT('Ctrl Pts',(-20.7451747360216,-17.3657046830186,
-18.6516819547758));
#59461=CARTESIAN_POINT('Ctrl Pts',(-20.6890551911698,-17.2993175745231,
-18.6559981175153));
#59462=CARTESIAN_POINT('Ctrl Pts',(-20.6347637346021,-17.23509301912,-18.6601736817065));
#59463=CARTESIAN_POINT('Ctrl Pts',(-20.5773433873059,-17.173592789127,-18.6643492458977));
#59464=CARTESIAN_POINT('Ctrl Pts',(-20.5171090485652,-17.1151216368728,
-18.668524810089));
#59465=CARTESIAN_POINT('Ctrl Pts',(-20.4538324165453,-17.0536972456979,
-18.6729112721026));
#59466=CARTESIAN_POINT('Ctrl Pts',(-20.3874504923529,-16.9956163559344,
-18.6772977341163));
#59467=CARTESIAN_POINT('Ctrl Pts',(-20.3183666557521,-16.9411836731962,
-18.6816841961299));
#59468=CARTESIAN_POINT('Ctrl Pts',(-20.2492828191514,-16.886750990458,-18.6860706581436));
#59469=CARTESIAN_POINT('Ctrl Pts',(-20.1774975877418,-16.835966787744,-18.6904571201572));
#59470=CARTESIAN_POINT('Ctrl Pts',(-20.1034462555221,-16.7890813808105,
-18.6948435821709));
#59471=CARTESIAN_POINT('Ctrl Pts',(-20.0328021348959,-16.7443532409684,
-18.6990282165633));
#59472=CARTESIAN_POINT('Ctrl Pts',(-19.9598329133702,-16.703006515634,-18.7032128509558));
#59473=CARTESIAN_POINT('Ctrl Pts',(-19.8848959073542,-16.665290877607,-18.7073974853483));
#59474=CARTESIAN_POINT('Ctrl Pts',(-19.810065564891,-16.6276289231225,-18.7115761634316));
#59475=CARTESIAN_POINT('Ctrl Pts',(-19.7332734088094,-16.5935879949175,
-18.715754841515));
#59476=CARTESIAN_POINT('Ctrl Pts',(-19.6549047742286,-16.5633739520798,
-18.7199335195983));
#59477=CARTESIAN_POINT('Ctrl Pts',(-19.5751314381813,-16.5326183442331,
-18.7241870974839));
#59478=CARTESIAN_POINT('Ctrl Pts',(-19.4937249583385,-16.5058284229433,
-18.7284406753695));
#59479=CARTESIAN_POINT('Ctrl Pts',(-19.4111169976704,-16.4831718222068,
-18.7326942532551));
#59480=CARTESIAN_POINT('Ctrl Pts',(-19.3301105535306,-16.4609544638903,
-18.7368653672324));
#59481=CARTESIAN_POINT('Ctrl Pts',(-19.247949263021,-16.4427117186153,-18.7410364812098));
#59482=CARTESIAN_POINT('Ctrl Pts',(-19.1650575928263,-16.4285520905581,
-18.7452075951871));
#59483=CARTESIAN_POINT('Ctrl Pts',(-19.0821937377322,-16.4143972139008,
-18.7493773095069));
#59484=CARTESIAN_POINT('Ctrl Pts',(-18.9986004427846,-16.4043228107593,
-18.7535470238266));
#59485=CARTESIAN_POINT('Ctrl Pts',(-18.9147123478962,-16.3983862767995,
-18.7577167381464));
#59486=CARTESIAN_POINT('Ctrl Pts',(-18.8308272381063,-16.3924499540871,
-18.7618863040898));
#59487=CARTESIAN_POINT('Ctrl Pts',(-18.7466478081782,-16.3906512394234,
-18.7660558700333));
#59488=CARTESIAN_POINT('Ctrl Pts',(-18.6626124310835,-16.3929955422071,
-18.7702254359767));
#59489=CARTESIAN_POINT('Ctrl Pts',(-18.5756224737719,-16.3954222677853,
-18.7745415987163));
#59490=CARTESIAN_POINT('Ctrl Pts',(-18.4887874147824,-16.4022887536938,
-18.778857761456));
#59491=CARTESIAN_POINT('Ctrl Pts',(-18.4025899172854,-16.4135423271059,
-18.7831739241956));
#59492=CARTESIAN_POINT('Ctrl Pts',(-18.319200294229,-16.4244293165443,-18.7873494883867));
#59493=CARTESIAN_POINT('Ctrl Pts',(-18.2364077885012,-16.439421833601,-18.7915250525778));
#59494=CARTESIAN_POINT('Ctrl Pts',(-18.1546390975922,-16.4584200544676,
-18.7957006167688));
#59495=CARTESIAN_POINT('Ctrl Pts',(-18.0687404644525,-16.4783778303154,
-18.8000870787827));
#59496=CARTESIAN_POINT('Ctrl Pts',(-17.9839723511228,-16.5027564393572,
-18.8044735407966));
#59497=CARTESIAN_POINT('Ctrl Pts',(-17.9008093086194,-16.5313816344172,
-18.8088600028106));
#59498=CARTESIAN_POINT('Ctrl Pts',(-17.8176462661159,-16.5600068294773,
-18.8132464648245));
#59499=CARTESIAN_POINT('Ctrl Pts',(-17.7360888041544,-16.5928783231054,
-18.8176329268384));
#59500=CARTESIAN_POINT('Ctrl Pts',(-17.6565830150583,-16.6297655931067,
-18.8220193888523));
#59501=CARTESIAN_POINT('Ctrl Pts',(-17.5807293782487,-16.6649584213697,
-18.8262043557618));
#59502=CARTESIAN_POINT('Ctrl Pts',(-17.5064606949899,-16.7039371893241,
-18.8303893226713));
#59503=CARTESIAN_POINT('Ctrl Pts',(-17.4341804046549,-16.7465365522057,
-18.8345742895809));
#59504=CARTESIAN_POINT('Ctrl Pts',(-17.3620114351116,-16.7890703066789,
-18.8387528111119));
#59505=CARTESIAN_POINT('Ctrl Pts',(-17.2918251656929,-16.8352133429876,
-18.8429313326429));
#59506=CARTESIAN_POINT('Ctrl Pts',(-17.2240032216123,-16.8847531039426,
-18.8471098541739));
#59507=CARTESIAN_POINT('Ctrl Pts',(-17.207345883423,-16.8969202655189,-18.848136115618));
#59508=CARTESIAN_POINT('Ctrl Pts',(-17.1908310530321,-16.9092921023112,
-18.8491623770621));
#59509=CARTESIAN_POINT('Ctrl Pts',(-17.1744641548914,-16.9218650419685,
-18.8501886385061));
#59510=CARTESIAN_POINT('Ctrl Pts',(-17.1744641548914,-16.9218650419685,
-18.0500683176022));
#59511=CARTESIAN_POINT('Ctrl Pts',(-17.1273611601948,-16.9580492416202,
-18.0530337279894));
#59512=CARTESIAN_POINT('Ctrl Pts',(-17.0815714136153,-16.9958326841265,
-18.0559991383765));
#59513=CARTESIAN_POINT('Ctrl Pts',(-17.03720428459,-17.0351055584185,-18.0589645487636));
#59514=CARTESIAN_POINT('Ctrl Pts',(-16.9745956774142,-17.0905254157143,
-18.0631491831567));
#59515=CARTESIAN_POINT('Ctrl Pts',(-16.9145885551718,-17.1491189671382,
-18.0673338175499));
#59516=CARTESIAN_POINT('Ctrl Pts',(-16.8575221052052,-17.2106124181141,
-18.071518451943));
#59517=CARTESIAN_POINT('Ctrl Pts',(-16.8005368822667,-17.2720183407739,
-18.075697130027));
#59518=CARTESIAN_POINT('Ctrl Pts',(-16.7464843277719,-17.3363156298582,
-18.079875808111));
#59519=CARTESIAN_POINT('Ctrl Pts',(-16.6956693348428,-17.4031913935286,
-18.084054486195));
#59520=CARTESIAN_POINT('Ctrl Pts',(-16.6439435196865,-17.4712658571988,
-18.0883080640804));
#59521=CARTESIAN_POINT('Ctrl Pts',(-16.5955728353228,-17.5420118234209,
-18.0925616419658));
#59522=CARTESIAN_POINT('Ctrl Pts',(-16.5508383402301,-17.6150612701733,
-18.0968152198512));
#59523=CARTESIAN_POINT('Ctrl Pts',(-16.5069711106161,-17.6866945108574,
-18.1009863338293));
#59524=CARTESIAN_POINT('Ctrl Pts',(-16.4666005905003,-17.7605423037905,
-18.1051574478073));
#59525=CARTESIAN_POINT('Ctrl Pts',(-16.4299490395872,-17.836227096663,-18.1093285617853));
#59526=CARTESIAN_POINT('Ctrl Pts',(-16.3933097874561,-17.9118864927724,
-18.1134982761057));
#59527=CARTESIAN_POINT('Ctrl Pts',(-16.3603872264447,-17.989381250901,-18.1176679904261));
#59528=CARTESIAN_POINT('Ctrl Pts',(-16.331357352511,-18.0683098345761,-18.1218377047466));
#59529=CARTESIAN_POINT('Ctrl Pts',(-16.3023285115847,-18.1472356096334,
-18.1260072706907));
#59530=CARTESIAN_POINT('Ctrl Pts',(-16.2771922403253,-18.227594676743,-18.1301768366348));
#59531=CARTESIAN_POINT('Ctrl Pts',(-16.2560756369329,-18.3089674573409,
-18.1343464025789));
#59532=CARTESIAN_POINT('Ctrl Pts',(-16.2342165998161,-18.393201204518,-18.1386625653177));
#59533=CARTESIAN_POINT('Ctrl Pts',(-16.2166652853052,-18.478520765314,-18.1429787280566));
#59534=CARTESIAN_POINT('Ctrl Pts',(-16.203505316394,-18.5644478664209,-18.1472948907955));
#59535=CARTESIAN_POINT('Ctrl Pts',(-16.1907740320855,-18.6475759012497,
-18.1514704549872));
#59536=CARTESIAN_POINT('Ctrl Pts',(-16.1821523920334,-18.7312720295791,
-18.1556460191789));
#59537=CARTESIAN_POINT('Ctrl Pts',(-16.177663165104,-18.8150986247193,-18.1598215833707));
#59538=CARTESIAN_POINT('Ctrl Pts',(-16.1729471979947,-18.9031591018972,
-18.1642080453831));
#59539=CARTESIAN_POINT('Ctrl Pts',(-16.172792072363,-18.9913629881318,-18.1685945073955));
#59540=CARTESIAN_POINT('Ctrl Pts',(-16.1771623761344,-19.0792059950832,
-18.1729809694079));
#59541=CARTESIAN_POINT('Ctrl Pts',(-16.1815326799057,-19.1670490020346,
-18.1773674314203));
#59542=CARTESIAN_POINT('Ctrl Pts',(-16.1904282787085,-19.2545305601574,
-18.1817538934327));
#59543=CARTESIAN_POINT('Ctrl Pts',(-16.2037517912765,-19.3411580684653,
-18.1861403554451));
#59544=CARTESIAN_POINT('Ctrl Pts',(-16.2164622692813,-19.4237997167046,
-18.1903249898381));
#59545=CARTESIAN_POINT('Ctrl Pts',(-16.2332494562529,-19.5059717882466,
-18.1945096242311));
#59546=CARTESIAN_POINT('Ctrl Pts',(-16.2540667299572,-19.5872408804027,
-18.1986942586241));
#59547=CARTESIAN_POINT('Ctrl Pts',(-16.274854372849,-19.6683942960652,-18.202872936708));
#59548=CARTESIAN_POINT('Ctrl Pts',(-16.299660595141,-19.748646843478,-18.2070516147919));
#59549=CARTESIAN_POINT('Ctrl Pts',(-16.3283873371777,-19.8275727933582,
-18.2112302928758));
#59550=CARTESIAN_POINT('Ctrl Pts',(-16.3576289854203,-19.9079134341682,
-18.2154838707612));
#59551=CARTESIAN_POINT('Ctrl Pts',(-16.3909330131977,-19.9868789746049,
-18.2197374486466));
#59552=CARTESIAN_POINT('Ctrl Pts',(-16.428142103854,-20.0640338856262,-18.2239910265321));
#59553=CARTESIAN_POINT('Ctrl Pts',(-16.4646298236797,-20.1396929981407,
-18.22816214051));
#59554=CARTESIAN_POINT('Ctrl Pts',(-16.5048723340172,-20.2136106264637,
-18.2323332544879));
#59555=CARTESIAN_POINT('Ctrl Pts',(-16.5486724780857,-20.2853955234528,
-18.2365043684658));
#59556=CARTESIAN_POINT('Ctrl Pts',(-16.5924579245929,-20.3571563323264,
-18.2406740827861));
#59557=CARTESIAN_POINT('Ctrl Pts',(-16.6397983945163,-20.4267854387981,
-18.2448437971064));
#59558=CARTESIAN_POINT('Ctrl Pts',(-16.6904515225008,-20.4939175140423,
-18.2490135114267));
#59559=CARTESIAN_POINT('Ctrl Pts',(-16.7411028480295,-20.5610472004393,
-18.2531830773707));
#59560=CARTESIAN_POINT('Ctrl Pts',(-16.795066319483,-20.6256796655625,-18.2573526433147));
#59561=CARTESIAN_POINT('Ctrl Pts',(-16.8520579335337,-20.6874809300205,
-18.2615222092587));
#59562=CARTESIAN_POINT('Ctrl Pts',(-16.9110533024294,-20.7514550506984,
-18.2658383719977));
#59563=CARTESIAN_POINT('Ctrl Pts',(-16.9732933572893,-20.8123947886944,
-18.2701545347367));
#59564=CARTESIAN_POINT('Ctrl Pts',(-17.0384212094901,-20.8699709500337,
-18.2744706974756));
#59565=CARTESIAN_POINT('Ctrl Pts',(-17.101427528754,-20.9256715739717,-18.2786462616673));
#59566=CARTESIAN_POINT('Ctrl Pts',(-17.1671359972395,-20.9782241356928,
-18.2828218258589));
#59567=CARTESIAN_POINT('Ctrl Pts',(-17.2351909645118,-21.0273726111566,
-18.2869973900505));
#59568=CARTESIAN_POINT('Ctrl Pts',(-17.3066832263984,-21.0790034592786,
-18.2913838520632));
#59569=CARTESIAN_POINT('Ctrl Pts',(-17.3807647695956,-21.1268769860888,
-18.2957703140758));
#59570=CARTESIAN_POINT('Ctrl Pts',(-17.4569923995305,-21.1707500058238,
-18.3001567760885));
#59571=CARTESIAN_POINT('Ctrl Pts',(-17.5332200294655,-21.2146230255589,
-18.3045432381011));
#59572=CARTESIAN_POINT('Ctrl Pts',(-17.6115931945078,-21.25449534292,-18.3089297001138));
#59573=CARTESIAN_POINT('Ctrl Pts',(-17.6916449845513,-21.2901822045702,
-18.3133161621265));
#59574=CARTESIAN_POINT('Ctrl Pts',(-17.7680134730656,-21.3242270608135,
-18.3175007965194));
#59575=CARTESIAN_POINT('Ctrl Pts',(-17.8461937671324,-21.3545898770089,
-18.3216854309123));
#59576=CARTESIAN_POINT('Ctrl Pts',(-17.9257962079471,-21.3810752624222,
-18.3258700653053));
#59577=CARTESIAN_POINT('Ctrl Pts',(-18.00528534454,-21.4075229491675,-18.3300487433891));
#59578=CARTESIAN_POINT('Ctrl Pts',(-18.0861921743113,-21.4301040236941,
-18.3342274214729));
#59579=CARTESIAN_POINT('Ctrl Pts',(-18.1681056484757,-21.4486704994678,
-18.3384060995568));
#59580=CARTESIAN_POINT('Ctrl Pts',(-18.2514873627971,-21.4675697659769,
-18.3426596774422));
#59581=CARTESIAN_POINT('Ctrl Pts',(-18.3359117243118,-21.4823088984315,
-18.3469132553277));
#59582=CARTESIAN_POINT('Ctrl Pts',(-18.4209273694976,-21.4927844316333,
-18.3511668332132));
#59583=CARTESIAN_POINT('Ctrl Pts',(-18.5042948205043,-21.5030568761823,
-18.355337947191));
#59584=CARTESIAN_POINT('Ctrl Pts',(-18.5882303557905,-21.5092295037566,
-18.3595090611688));
#59585=CARTESIAN_POINT('Ctrl Pts',(-18.6722982811997,-21.5112563173502,
-18.3636801751467));
#59586=CARTESIAN_POINT('Ctrl Pts',(-18.7563379968047,-21.513282450827,-18.3678498894669));
#59587=CARTESIAN_POINT('Ctrl Pts',(-18.8405095547877,-21.5111655221263,
-18.3720196037872));
#59588=CARTESIAN_POINT('Ctrl Pts',(-18.9243745836512,-21.5049115765924,
-18.3761893181074));
#59589=CARTESIAN_POINT('Ctrl Pts',(-19.0082366282371,-21.4986578536008,
-18.3803588840514));
#59590=CARTESIAN_POINT('Ctrl Pts',(-19.0917917066947,-21.4882674415331,
-18.3845284499953));
#59591=CARTESIAN_POINT('Ctrl Pts',(-19.1746052695949,-21.4737983655331,
-18.3886980159392));
#59592=CARTESIAN_POINT('Ctrl Pts',(-19.2603304552103,-21.4588205746695,
-18.3930141786783));
#59593=CARTESIAN_POINT('Ctrl Pts',(-19.3452604921636,-21.4394720625983,
-18.3973303414173));
#59594=CARTESIAN_POINT('Ctrl Pts',(-19.4289254033755,-21.4158747297181,
-18.4016465041564));
#59595=CARTESIAN_POINT('Ctrl Pts',(-19.5098649388997,-21.3930460774758,
-18.405822068348));
#59596=CARTESIAN_POINT('Ctrl Pts',(-19.5896200744146,-21.3662413589924,
-18.4099976325395));
#59597=CARTESIAN_POINT('Ctrl Pts',(-19.6677830273837,-21.3356210390434,
-18.4141731967311));
#59598=CARTESIAN_POINT('Ctrl Pts',(-19.7498938052998,-21.3034541595237,
-18.4185596587439));
#59599=CARTESIAN_POINT('Ctrl Pts',(-19.8302467994653,-21.2670763374215,
-18.4229461207567));
#59600=CARTESIAN_POINT('Ctrl Pts',(-19.9083976363218,-21.2267285973939,
-18.4273325827695));
#59601=CARTESIAN_POINT('Ctrl Pts',(-19.9865484731783,-21.1863808573664,
-18.4317190447823));
#59602=CARTESIAN_POINT('Ctrl Pts',(-20.0624966899234,-21.1420635575359,
-18.4361055067951));
#59603=CARTESIAN_POINT('Ctrl Pts',(-20.1358342086536,-21.0940692919344,
-18.4404919688079));
#59604=CARTESIAN_POINT('Ctrl Pts',(-20.2057039471169,-21.0483444454524,
-18.4446710160258));
#59605=CARTESIAN_POINT('Ctrl Pts',(-20.2734659150701,-20.9991112651902,
-18.4488500632436));
#59606=CARTESIAN_POINT('Ctrl Pts',(-20.3387454860835,-20.9465906660001,
-18.4530291104615));
#59607=CARTESIAN_POINT('Ctrl Pts',(-20.4039320790896,-20.8941448721524,
-18.4572022054423));
#59608=CARTESIAN_POINT('Ctrl Pts',(-20.46664294125,-20.8384212459577,-18.461375300423));
#59609=CARTESIAN_POINT('Ctrl Pts',(-20.5265316718116,-20.7796843834624,
-18.4655483954038));
#59610=CARTESIAN_POINT('Ctrl Pts',(-20.5870226816093,-20.7203568256503,
-18.4697634576868));
#59611=CARTESIAN_POINT('Ctrl Pts',(-20.6446340707897,-20.6579553356914,
-18.4739785199699));
#59612=CARTESIAN_POINT('Ctrl Pts',(-20.6990425114804,-20.5927949073771,
-18.4781935822529));
#59613=CARTESIAN_POINT('Ctrl Pts',(-20.7528122887531,-20.528399352699,-18.4823591668069));
#59614=CARTESIAN_POINT('Ctrl Pts',(-20.803453612438,-20.4613096522777,-18.4865247513609));
#59615=CARTESIAN_POINT('Ctrl Pts',(-20.8506921231955,-20.3918661241943,
-18.4906903359149));
#59616=CARTESIAN_POINT('Ctrl Pts',(-20.8979149500345,-20.3224456524396,
-18.4948545374302));
#59617=CARTESIAN_POINT('Ctrl Pts',(-20.9417369482816,-20.2506732862343,
-18.4990187389455));
#59618=CARTESIAN_POINT('Ctrl Pts',(-20.9819260328718,-20.1769198140031,
-18.5031829404608));
#59619=CARTESIAN_POINT('Ctrl Pts',(-21.0221139173366,-20.1031685441961,
-18.5073470176248));
#59620=CARTESIAN_POINT('Ctrl Pts',(-21.0586688839111,-20.0274366916314,
-18.5115110947889));
#59621=CARTESIAN_POINT('Ctrl Pts',(-21.0914046022627,-19.9501200034218,
-18.5156751719529));
#59622=CARTESIAN_POINT('Ctrl Pts',(-21.1248385440614,-19.8711542197507,
-18.5199280651399));
#59623=CARTESIAN_POINT('Ctrl Pts',(-21.1542882228969,-19.7905356687051,
-18.5241809583268));
#59624=CARTESIAN_POINT('Ctrl Pts',(-21.1796074785074,-19.7087060598863,
-18.5284338515138));
#59625=CARTESIAN_POINT('Ctrl Pts',(-21.2044336791703,-19.6284699613236,
-18.5326039259141));
#59626=CARTESIAN_POINT('Ctrl Pts',(-21.2252888283687,-19.5470700198229,
-18.5367740003145));
#59627=CARTESIAN_POINT('Ctrl Pts',(-21.2420864983913,-19.4649348073461,
-18.5409440747148));
#59628=CARTESIAN_POINT('Ctrl Pts',(-21.2593845777048,-19.3803527541243,
-18.5452383772951));
#59629=CARTESIAN_POINT('Ctrl Pts',(-21.2723795196075,-19.294991452669,-18.5495326798753));
#59630=CARTESIAN_POINT('Ctrl Pts',(-21.2810343673868,-19.2093245642189,
-18.5538269824556));
#59631=CARTESIAN_POINT('Ctrl Pts',(-21.2896892151661,-19.1236576757689,
-18.5581212850359));
#59632=CARTESIAN_POINT('Ctrl Pts',(-21.2940040128973,-19.0376857298059,
-18.5624155876161));
#59633=CARTESIAN_POINT('Ctrl Pts',(-21.2939999971965,-18.9518801919504,
-18.5667098901964));
#59634=CARTESIAN_POINT('Origin',(-18.734,-18.952,1.76670989022851));
#59635=CARTESIAN_POINT('',(-17.1762220723152,-16.9241895431829,-17.2500265390144));
#59636=CARTESIAN_POINT('',(-17.1735447326512,-16.9206895600705,-17.3168006994722));
#59637=CARTESIAN_POINT('',(-17.1744641548914,-16.9218650419685,1.76670989022851));
#59638=CARTESIAN_POINT('',(-21.2939989159607,-18.9543559031924,-17.8332901097715));
#59639=CARTESIAN_POINT('Ctrl Pts',(-17.1735447326512,-16.9206895600706,
-17.3168006994722));
#59640=CARTESIAN_POINT('Ctrl Pts',(-16.6213792717057,-17.3535717521052,
-17.3517574528043));
#59641=CARTESIAN_POINT('Ctrl Pts',(-15.7867861609283,-18.831728284438,-17.4291061416968));
#59642=CARTESIAN_POINT('Ctrl Pts',(-16.8703561902843,-21.337397809626,-17.5488467661498));
#59643=CARTESIAN_POINT('Ctrl Pts',(-19.7309870131108,-21.8102001076479,
-17.6760225728312));
#59644=CARTESIAN_POINT('Ctrl Pts',(-21.1817725818657,-20.2077259866878,
-17.7708370079975));
#59645=CARTESIAN_POINT('Ctrl Pts',(-21.2957663888719,-19.1559927477998,
-17.8232595076033));
#59646=CARTESIAN_POINT('Ctrl Pts',(-21.2939116922138,-18.9543565892689,
-17.8332900716486));
#59647=CARTESIAN_POINT('Ctrl Pts',(-21.2939989159607,-18.9543559031924,
-17.8332901097715));
#59648=CARTESIAN_POINT('Ctrl Pts',(-21.2940751741219,-18.8714913735434,
-17.837412174938));
#59649=CARTESIAN_POINT('Ctrl Pts',(-21.290123839502,-18.7885152466555,-17.8415342401044));
#59650=CARTESIAN_POINT('Ctrl Pts',(-21.2821391268744,-18.7058557534859,
-17.8456563052709));
#59651=CARTESIAN_POINT('Ctrl Pts',(-21.2741597741335,-18.6232517470386,
-17.8497756034244));
#59652=CARTESIAN_POINT('Ctrl Pts',(-21.262152459652,-18.5409644216312,-17.8538949015779));
#59653=CARTESIAN_POINT('Ctrl Pts',(-21.2461634417033,-18.4594202174576,
-17.8580141997315));
#59654=CARTESIAN_POINT('Ctrl Pts',(-21.2301800733889,-18.3779048264943,
-17.862132042353));
#59655=CARTESIAN_POINT('Ctrl Pts',(-21.2102178848107,-18.2971324990613,
-17.8662498849744));
#59656=CARTESIAN_POINT('Ctrl Pts',(-21.1863745538874,-18.217521240984,-17.8703677275959));
#59657=CARTESIAN_POINT('Ctrl Pts',(-21.1625320679642,-18.1379128043046,
-17.8744854242823));
#59658=CARTESIAN_POINT('Ctrl Pts',(-21.1348088500427,-18.0594658076282,
-17.8786031209688));
#59659=CARTESIAN_POINT('Ctrl Pts',(-21.103352505349,-17.9825833169393,-17.8827208176552));
#59660=CARTESIAN_POINT('Ctrl Pts',(-21.071866121991,-17.905627408714,-17.8868424464612));
#59661=CARTESIAN_POINT('Ctrl Pts',(-21.0366396717683,-17.8302394286303,
-17.8909640752672));
#59662=CARTESIAN_POINT('Ctrl Pts',(-20.9978687619911,-17.7568020128526,
-17.8950857040732));
#59663=CARTESIAN_POINT('Ctrl Pts',(-20.9590794967265,-17.683329829267,-17.8992092842005));
#59664=CARTESIAN_POINT('Ctrl Pts',(-20.9167426732498,-17.6118104548626,
-17.9033328643279));
#59665=CARTESIAN_POINT('Ctrl Pts',(-20.8710983794442,-17.5425992349311,
-17.9074564444553));
#59666=CARTESIAN_POINT('Ctrl Pts',(-20.8253741239691,-17.4732667677585,
-17.9115872484506));
#59667=CARTESIAN_POINT('Ctrl Pts',(-20.776331105883,-17.4062509123682,-17.9157180524459));
#59668=CARTESIAN_POINT('Ctrl Pts',(-20.724250792007,-17.3418752269108,-17.9198488564413));
#59669=CARTESIAN_POINT('Ctrl Pts',(-20.6800170723894,-17.2871985975131,
-17.9233572996922));
#59670=CARTESIAN_POINT('Ctrl Pts',(-20.6335931281536,-17.2344260450368,
-17.9268657429431));
#59671=CARTESIAN_POINT('Ctrl Pts',(-20.5851713910723,-17.1837340469049,
-17.930374186194));
#59672=CARTESIAN_POINT('Ctrl Pts',(-20.5274172101246,-17.1232720517519,
-17.934558820587));
#59673=CARTESIAN_POINT('Ctrl Pts',(-20.4665902688467,-17.0655300202436,
-17.93874345498));
#59674=CARTESIAN_POINT('Ctrl Pts',(-20.4029770272298,-17.0108365131759,
-17.942928089373));
#59675=CARTESIAN_POINT('Ctrl Pts',(-20.3394543311885,-16.9562208555457,
-17.9471067674569));
#59676=CARTESIAN_POINT('Ctrl Pts',(-20.2731535582845,-16.9046454006956,
-17.9512854455408));
#59677=CARTESIAN_POINT('Ctrl Pts',(-20.2043989371765,-16.8564029572577,
-17.9554641236247));
#59678=CARTESIAN_POINT('Ctrl Pts',(-20.1344119388971,-16.8072958026916,
-17.9597177015102));
#59679=CARTESIAN_POINT('Ctrl Pts',(-20.0618825897098,-16.7616426719214,
-17.9639712793956));
#59680=CARTESIAN_POINT('Ctrl Pts',(-19.9871893049686,-16.7197104654834,
-17.9682248572811));
#59681=CARTESIAN_POINT('Ctrl Pts',(-19.9139440953053,-16.6785911966919,
-17.972395971259));
#59682=CARTESIAN_POINT('Ctrl Pts',(-19.8386185251852,-16.6410501005271,
-17.9765670852369));
#59683=CARTESIAN_POINT('Ctrl Pts',(-19.7615983036834,-16.6072949596448,
-17.9807381992148));
#59684=CARTESIAN_POINT('Ctrl Pts',(-19.6846039270608,-16.5735511456261,
-17.9849079135351));
#59685=CARTESIAN_POINT('Ctrl Pts',(-19.6059164494112,-16.5435909483339,
-17.9890776278554));
#59686=CARTESIAN_POINT('Ctrl Pts',(-19.5259437923519,-16.517575010448,-17.9932473421758));
#59687=CARTESIAN_POINT('Ctrl Pts',(-19.4459739810629,-16.4915599983208,
-17.9974169081197));
#59688=CARTESIAN_POINT('Ctrl Pts',(-19.3647195190222,-16.469489108043,-18.0015864740637));
#59689=CARTESIAN_POINT('Ctrl Pts',(-19.2826045027056,-16.4514734355318,
-18.0057560400077));
#59690=CARTESIAN_POINT('Ctrl Pts',(-19.1976024237126,-16.4328243541993,
-18.0100722027467));
#59691=CARTESIAN_POINT('Ctrl Pts',(-19.1116786655145,-16.4185210722996,
-18.0143883654857));
#59692=CARTESIAN_POINT('Ctrl Pts',(-19.0253143284884,-16.4086290160464,
-18.0187045282247));
#59693=CARTESIAN_POINT('Ctrl Pts',(-18.9417633006593,-16.3990591924854,
-18.0228800924163));
#59694=CARTESIAN_POINT('Ctrl Pts',(-18.8578004300249,-16.3936175999791,
-18.0270556566079));
#59695=CARTESIAN_POINT('Ctrl Pts',(-18.7738638919265,-16.3923103957471,
-18.0312312207996));
#59696=CARTESIAN_POINT('Ctrl Pts',(-18.6856879188254,-16.3909371677368,
-18.0356176828122));
#59697=CARTESIAN_POINT('Ctrl Pts',(-18.5975415917828,-16.3941269389876,
-18.0400041448249));
#59698=CARTESIAN_POINT('Ctrl Pts',(-18.5099274935594,-16.4018251997447,
-18.0443906068376));
#59699=CARTESIAN_POINT('Ctrl Pts',(-18.4223133953359,-16.4095234605017,
-18.0487770688502));
#59700=CARTESIAN_POINT('Ctrl Pts',(-18.3352320899719,-16.4217300548923,
-18.0531635308629));
#59701=CARTESIAN_POINT('Ctrl Pts',(-18.249172131343,-16.4383289917387,-18.0575499928756));
#59702=CARTESIAN_POINT('Ctrl Pts',(-18.1670679985969,-16.4541649430451,
-18.0617348270901));
#59703=CARTESIAN_POINT('Ctrl Pts',(-18.0855877575642,-16.4740572520247,
-18.0659196613047));
#59704=CARTESIAN_POINT('Ctrl Pts',(-18.0051627929096,-16.4979428846173,
-18.0701044955193));
#59705=CARTESIAN_POINT('Ctrl Pts',(-17.9248712290264,-16.5217888981459,
-18.0742823883554));
#59706=CARTESIAN_POINT('Ctrl Pts',(-17.8456318987211,-16.5496149366924,
-18.0784602811916));
#59707=CARTESIAN_POINT('Ctrl Pts',(-17.7678662694262,-16.5813069336906,
-18.0826381740277));
#59708=CARTESIAN_POINT('Ctrl Pts',(-17.6901757083229,-16.6129683379845,
-18.0868120338886));
#59709=CARTESIAN_POINT('Ctrl Pts',(-17.6139564476478,-16.648488119702,-18.0909858937495));
#59710=CARTESIAN_POINT('Ctrl Pts',(-17.5396142320594,-16.6877026172914,
-18.0951597536104));
#59711=CARTESIAN_POINT('Ctrl Pts',(-17.4653211999375,-16.7268911712778,
-18.099330852121));
#59712=CARTESIAN_POINT('Ctrl Pts',(-17.392903152695,-16.7697693732504,-18.1035019506317));
#59713=CARTESIAN_POINT('Ctrl Pts',(-17.3227440412668,-16.8161262633433,
-18.1076730491423));
#59714=CARTESIAN_POINT('Ctrl Pts',(-17.2720952992043,-16.8495918834365,
-18.1106842174465));
#59715=CARTESIAN_POINT('Ctrl Pts',(-17.2226233973444,-16.8848694399857,
-18.1136953857507));
#59716=CARTESIAN_POINT('Ctrl Pts',(-17.1744641548915,-16.9218650419685,
-18.1167065540548));
#59717=CARTESIAN_POINT('',(-21.2939990418858,-18.9497851537328,-17.7667099127498));
#59718=CARTESIAN_POINT('Ctrl Pts',(-21.2939990418858,-18.9497851537328,
-17.7667099127498));
#59719=CARTESIAN_POINT('Ctrl Pts',(-21.2939112972755,-18.8483667746996,
-17.7717442924651));
#59720=CARTESIAN_POINT('Ctrl Pts',(-21.2877929815452,-18.7472123213116,
-17.7767786721804));
#59721=CARTESIAN_POINT('Ctrl Pts',(-21.275760552819,-18.64695362298,-17.7818130518957));
#59722=CARTESIAN_POINT('Ctrl Pts',(-21.2635573150894,-18.54527168012,-17.7869188982619));
#59723=CARTESIAN_POINT('Ctrl Pts',(-21.245270932926,-18.4445110968148,-17.792024744628));
#59724=CARTESIAN_POINT('Ctrl Pts',(-21.2210717431372,-18.345308855769,-17.7971305909941));
#59725=CARTESIAN_POINT('Ctrl Pts',(-21.2092508709201,-18.2968503319384,
-17.7996247057963));
#59726=CARTESIAN_POINT('Ctrl Pts',(-21.1960198419216,-18.2487633198847,
-17.8021188205986));
#59727=CARTESIAN_POINT('Ctrl Pts',(-21.1814026084241,-18.201120201178,-17.8046129354008));
#59728=CARTESIAN_POINT('Ctrl Pts',(-21.1568777637899,-18.121184412756,-17.8087975697939));
#59729=CARTESIAN_POINT('Ctrl Pts',(-21.1283869296254,-18.0423026572185,
-17.8129822041869));
#59730=CARTESIAN_POINT('Ctrl Pts',(-21.0960388974778,-17.9648970434641,
-17.8171668385799));
#59731=CARTESIAN_POINT('Ctrl Pts',(-21.0637369087501,-17.88760160702,-17.8213455166639));
#59732=CARTESIAN_POINT('Ctrl Pts',(-21.0275888032569,-17.8117785597318,
-17.8255241947478));
#59733=CARTESIAN_POINT('Ctrl Pts',(-20.9877531601769,-17.7378349811526,
-17.8297028728318));
#59734=CARTESIAN_POINT('Ctrl Pts',(-20.947203491824,-17.6625660170697,-17.8339564507172));
#59735=CARTESIAN_POINT('Ctrl Pts',(-20.9028329287837,-17.5892450243181,
-17.8382100286026));
#59736=CARTESIAN_POINT('Ctrl Pts',(-20.8548601014715,-17.5182802121801,
-17.8424636064881));
#59737=CARTESIAN_POINT('Ctrl Pts',(-20.8078173210281,-17.448691191402,-17.846634720466));
#59738=CARTESIAN_POINT('Ctrl Pts',(-20.7573109732373,-17.3813682068563,
-17.850805834444));
#59739=CARTESIAN_POINT('Ctrl Pts',(-20.7035927080245,-17.3166698912767,
-17.8549769484219));
#59740=CARTESIAN_POINT('Ctrl Pts',(-20.6498924684943,-17.2519932858418,
-17.8591466627423));
#59741=CARTESIAN_POINT('Ctrl Pts',(-20.5929827456749,-17.1899399538653,
-17.8633163770627));
#59742=CARTESIAN_POINT('Ctrl Pts',(-20.533156175962,-17.1308363460419,-17.867486091383));
#59743=CARTESIAN_POINT('Ctrl Pts',(-20.4733317351351,-17.0717348413785,
-17.8716556573271));
#59744=CARTESIAN_POINT('Ctrl Pts',(-20.4105909816463,-17.015583174876,-17.8758252232711));
#59745=CARTESIAN_POINT('Ctrl Pts',(-20.345263220069,-16.9626707573524,-17.8799947892152));
#59746=CARTESIAN_POINT('Ctrl Pts',(-20.2776386149851,-16.9078980045031,
-17.8843109519541));
#59747=CARTESIAN_POINT('Ctrl Pts',(-20.2072421084912,-16.8565968547186,
-17.888627114693));
#59748=CARTESIAN_POINT('Ctrl Pts',(-20.134474432863,-16.8090414462951,-17.8929432774319));
#59749=CARTESIAN_POINT('Ctrl Pts',(-20.0640771566148,-16.7630351502991,
-17.8971188416236));
#59750=CARTESIAN_POINT('Ctrl Pts',(-19.9914612509379,-16.7205345053977,
-17.9012944058153));
#59751=CARTESIAN_POINT('Ctrl Pts',(-19.9170156443953,-16.6817414276968,
-17.905469970007));
#59752=CARTESIAN_POINT('Ctrl Pts',(-19.8388099672436,-16.640989003863,-17.9098564320195));
#59753=CARTESIAN_POINT('Ctrl Pts',(-19.7585854263165,-16.604328771398,-17.9142428940321));
#59754=CARTESIAN_POINT('Ctrl Pts',(-19.6768157184724,-16.5719372863302,
-17.9186293560446));
#59755=CARTESIAN_POINT('Ctrl Pts',(-19.5950460106283,-16.5395458012623,
-17.9230158180572));
#59756=CARTESIAN_POINT('Ctrl Pts',(-19.5117317099373,-16.5114231770868,
-17.9274022800697));
#59757=CARTESIAN_POINT('Ctrl Pts',(-19.427361531773,-16.4876847226344,-17.9317887420823));
#59758=CARTESIAN_POINT('Ctrl Pts',(-19.3468694922175,-16.4650374240706,
-17.9359735770738));
#59759=CARTESIAN_POINT('Ctrl Pts',(-19.2651168916056,-16.446295797893,-17.9401584120653));
#59760=CARTESIAN_POINT('Ctrl Pts',(-19.1825176034853,-16.431596865705,-17.9443432470568));
#59761=CARTESIAN_POINT('Ctrl Pts',(-19.1000369486853,-16.4169190448749,
-17.9485220715744));
#59762=CARTESIAN_POINT('Ctrl Pts',(-19.0167124711285,-16.4062724641104,
-17.952700896092));
#59763=CARTESIAN_POINT('Ctrl Pts',(-18.9329723420367,-16.3997441336918,
-17.9568797206096));
#59764=CARTESIAN_POINT('Ctrl Pts',(-18.849333389066,-16.3932236909033,-17.9610534962066));
#59765=CARTESIAN_POINT('Ctrl Pts',(-18.7652802392365,-16.3908116415348,
-17.9652272718037));
#59766=CARTESIAN_POINT('Ctrl Pts',(-18.6812489272122,-16.392543549048,-17.9694010474007));
#59767=CARTESIAN_POINT('Ctrl Pts',(-18.5972730476301,-16.3942743140839,
-17.9735720697078));
#59768=CARTESIAN_POINT('Ctrl Pts',(-18.5133194358208,-16.4001435983923,
-17.9777430920148));
#59769=CARTESIAN_POINT('Ctrl Pts',(-18.4298258472946,-16.4101349200192,
-17.9819141143218));
#59770=CARTESIAN_POINT('Ctrl Pts',(-18.3463622898557,-16.4201226479539,
-17.9860836363899));
#59771=CARTESIAN_POINT('Ctrl Pts',(-18.2633588832482,-16.4342294129595,
-17.9902531584579));
#59772=CARTESIAN_POINT('Ctrl Pts',(-18.1812486084936,-16.4523868500931,
-17.994422680526));
#59773=CARTESIAN_POINT('Ctrl Pts',(-18.0991432365368,-16.4705432030475,
-17.9985919536322));
#59774=CARTESIAN_POINT('Ctrl Pts',(-18.0179313390458,-16.4927496461538,
-18.0027612267385));
#59775=CARTESIAN_POINT('Ctrl Pts',(-17.9380347007016,-16.5188869236485,
-18.0069304998447));
#59776=CARTESIAN_POINT('Ctrl Pts',(-17.8580775668942,-16.5450439915467,
-18.011102929806));
#59777=CARTESIAN_POINT('Ctrl Pts',(-17.7794381185581,-16.575137693535,-18.0152753597673));
#59778=CARTESIAN_POINT('Ctrl Pts',(-17.7025213244059,-16.6089994148967,
-18.0194477897286));
#59779=CARTESIAN_POINT('Ctrl Pts',(-17.6255715834959,-16.6428756406841,
-18.0236220069204));
#59780=CARTESIAN_POINT('Ctrl Pts',(-17.5503463787678,-16.6805228962677,
-18.0277962241122));
#59781=CARTESIAN_POINT('Ctrl Pts',(-17.4772271063916,-16.7217260495869,
-18.031970441304));
#59782=CARTESIAN_POINT('Ctrl Pts',(-17.4040091461644,-16.7629848141085,
-18.0361502923664));
#59783=CARTESIAN_POINT('Ctrl Pts',(-17.33290318242,-16.8078088135164,-18.0403301434289));
#59784=CARTESIAN_POINT('Ctrl Pts',(-17.2642621215538,-16.8559392736229,
-18.0445099944913));
#59785=CARTESIAN_POINT('Ctrl Pts',(-17.2338360617677,-16.877273737838,-18.0463627688616));
#59786=CARTESIAN_POINT('Ctrl Pts',(-17.2038938829713,-16.8992573253382,
-18.0482155432319));
#59787=CARTESIAN_POINT('Ctrl Pts',(-17.1744641548914,-16.9218650419685,
-18.0500683176022));
#59788=CARTESIAN_POINT('Ctrl Pts',(-17.1762220723153,-16.9241895431828,
-17.2500265390144));
#59789=CARTESIAN_POINT('Ctrl Pts',(-16.9304195468325,-17.1103102396675,
-17.2653209289013));
#59790=CARTESIAN_POINT('Ctrl Pts',(-16.1279941091616,-17.9709562098429,
-17.3230072543487));
#59791=CARTESIAN_POINT('Ctrl Pts',(-15.9988188303479,-20.2489482632501,
-17.4230855153565));
#59792=CARTESIAN_POINT('Ctrl Pts',(-18.3440265525621,-21.9538680082012,
-17.5502613220379));
#59793=CARTESIAN_POINT('Ctrl Pts',(-20.7784813047341,-21.0089843504267,
-17.6648027803286));
#59794=CARTESIAN_POINT('Ctrl Pts',(-21.2874612586096,-19.5488856065476,
-17.7369523030588));
#59795=CARTESIAN_POINT('Ctrl Pts',(-21.2923872581368,-18.9497870016169,
-17.7667098902285));
#59796=CARTESIAN_POINT('Origin',(-18.734,-18.952,1.76670989022851));
#59797=CARTESIAN_POINT('',(-17.1744641548914,-16.9218650419685,-16.4501666890971));
#59798=CARTESIAN_POINT('',(-17.1744641548915,-16.9218650419685,-16.5166303545479));
#59799=CARTESIAN_POINT('',(-17.1744641548914,-16.9218650419685,1.76670989022851));
#59800=CARTESIAN_POINT('',(-21.2942629985695,-18.9511644346814,-17.0332901097715));
#59801=CARTESIAN_POINT('Ctrl Pts',(-17.1744641548915,-16.9218650419685,
-16.5166303545479));
#59802=CARTESIAN_POINT('Ctrl Pts',(-17.1078974490003,-16.9730011319695,
-16.520815184908));
#59803=CARTESIAN_POINT('Ctrl Pts',(-17.0439434077443,-17.0273416600971,
-16.5250000152682));
#59804=CARTESIAN_POINT('Ctrl Pts',(-16.9829077605317,-17.0845750433086,
-16.5291848456283));
#59805=CARTESIAN_POINT('Ctrl Pts',(-16.9719424500703,-17.0948572610671,
-16.529936667985));
#59806=CARTESIAN_POINT('Ctrl Pts',(-16.9610712293328,-17.1052327594906,
-16.5306884903417));
#59807=CARTESIAN_POINT('Ctrl Pts',(-16.9502957329766,-17.115699619397,-16.5314403126983));
#59808=CARTESIAN_POINT('Ctrl Pts',(-16.8903194470162,-17.1739580385086,
-16.5356249470914));
#59809=CARTESIAN_POINT('Ctrl Pts',(-16.8330887583091,-17.2352663353223,
-16.5398095814844));
#59810=CARTESIAN_POINT('Ctrl Pts',(-16.7789298175348,-17.2993353087708,
-16.5439942158775));
#59811=CARTESIAN_POINT('Ctrl Pts',(-16.7248479653093,-17.3633130879657,
-16.5481728939614));
#59812=CARTESIAN_POINT('Ctrl Pts',(-16.6738294707906,-17.4300433902868,
-16.5523515720454));
#59813=CARTESIAN_POINT('Ctrl Pts',(-16.6261644175018,-17.4991995466843,
-16.5565302501293));
#59814=CARTESIAN_POINT('Ctrl Pts',(-16.577645002389,-17.5695952774836,-16.5607838280147));
#59815=CARTESIAN_POINT('Ctrl Pts',(-16.5326007777018,-17.6425043486949,
-16.5650374059002));
#59816=CARTESIAN_POINT('Ctrl Pts',(-16.4912954660574,-17.7175461234078,
-16.5692909837856));
#59817=CARTESIAN_POINT('Ctrl Pts',(-16.45079093848,-17.791133066886,-16.5734620977636));
#59818=CARTESIAN_POINT('Ctrl Pts',(-16.4138818774499,-17.8667703369927,
-16.5776332117415));
#59819=CARTESIAN_POINT('Ctrl Pts',(-16.3807728287042,-17.9440704983605,
-16.5818043257195));
#59820=CARTESIAN_POINT('Ctrl Pts',(-16.3476748900196,-18.0213447209125,
-16.5859740400399));
#59821=CARTESIAN_POINT('Ctrl Pts',(-16.318374612164,-18.1002803040064,-16.5901437543602));
#59822=CARTESIAN_POINT('Ctrl Pts',(-16.2930292165598,-18.1804679952255,
-16.5943134686806));
#59823=CARTESIAN_POINT('Ctrl Pts',(-16.2676847228536,-18.2606528330224,
-16.5984830346246));
#59824=CARTESIAN_POINT('Ctrl Pts',(-16.2462949694201,-18.3420892514569,
-16.6026526005687));
#59825=CARTESIAN_POINT('Ctrl Pts',(-16.2289674972205,-18.4243522386873,
-16.6068221665127));
#59826=CARTESIAN_POINT('Ctrl Pts',(-16.2110308124741,-18.5095074910663,
-16.6111383292517));
#59827=CARTESIAN_POINT('Ctrl Pts',(-16.1974474922546,-18.5955480019176,
-16.6154544919906));
#59828=CARTESIAN_POINT('Ctrl Pts',(-16.1882789321129,-18.6819921399002,
-16.6197706547295));
#59829=CARTESIAN_POINT('Ctrl Pts',(-16.1794090368535,-18.7656203691804,
-16.6239462189212));
#59830=CARTESIAN_POINT('Ctrl Pts',(-16.1746706763875,-18.8496258601583,
-16.6281217831129));
#59831=CARTESIAN_POINT('Ctrl Pts',(-16.1740663387713,-18.9335704012975,
-16.6322973473045));
#59832=CARTESIAN_POINT('Ctrl Pts',(-16.1734314774988,-19.0217547816503,
-16.6366838093171));
#59833=CARTESIAN_POINT('Ctrl Pts',(-16.1773592072922,-19.1098713098955,
-16.6410702713296));
#59834=CARTESIAN_POINT('Ctrl Pts',(-16.1857908120614,-19.1974178773141,
-16.6454567333422));
#59835=CARTESIAN_POINT('Ctrl Pts',(-16.1942224168306,-19.2849644447327,
-16.6498431953547));
#59836=CARTESIAN_POINT('Ctrl Pts',(-16.2071577359856,-19.3719404886095,
-16.6542296573672));
#59837=CARTESIAN_POINT('Ctrl Pts',(-16.2244766916358,-19.4578584434176,
-16.6586161193798));
#59838=CARTESIAN_POINT('Ctrl Pts',(-16.2409987764638,-19.5398231857641,
-16.6628007537728));
#59839=CARTESIAN_POINT('Ctrl Pts',(-16.2615714655045,-19.6211301562753,
-16.6669853881659));
#59840=CARTESIAN_POINT('Ctrl Pts',(-16.2861281256043,-19.7013485747917,
-16.6711700225589));
#59841=CARTESIAN_POINT('Ctrl Pts',(-16.3106498323379,-19.7814528123184,
-16.6753487006429));
#59842=CARTESIAN_POINT('Ctrl Pts',(-16.3391441128499,-19.8604711393629,
-16.6795273787268));
#59843=CARTESIAN_POINT('Ctrl Pts',(-16.3714933068752,-19.9379828218282,
-16.6837060568108));
#59844=CARTESIAN_POINT('Ctrl Pts',(-16.4044223369544,-20.0168838454952,
-16.6879596346962));
#59845=CARTESIAN_POINT('Ctrl Pts',(-16.4413457432406,-20.0942232074709,
-16.6922132125816));
#59846=CARTESIAN_POINT('Ctrl Pts',(-16.48208621838,-20.1695731272288,-16.6964667904671));
#59847=CARTESIAN_POINT('Ctrl Pts',(-16.5220368599103,-20.2434622417589,
-16.700637904445));
#59848=CARTESIAN_POINT('Ctrl Pts',(-16.5656576595127,-20.3154379408342,
-16.704809018423));
#59849=CARTESIAN_POINT('Ctrl Pts',(-16.6127335620839,-20.3851185224435,
-16.7089801324009));
#59850=CARTESIAN_POINT('Ctrl Pts',(-16.6597936678814,-20.4547757220608,
-16.7131498467213));
#59851=CARTESIAN_POINT('Ctrl Pts',(-16.7103063167569,-20.5221389528648,
-16.7173195610417));
#59852=CARTESIAN_POINT('Ctrl Pts',(-16.7640124931678,-20.5868544959491,
-16.721489275362));
#59853=CARTESIAN_POINT('Ctrl Pts',(-16.8177167584824,-20.6515677361767,
-16.7256588413061));
#59854=CARTESIAN_POINT('Ctrl Pts',(-16.8746140309484,-20.713633122547,-16.7298284072501));
#59855=CARTESIAN_POINT('Ctrl Pts',(-16.934405152749,-20.7727301792818,-16.7339979731942));
#59856=CARTESIAN_POINT('Ctrl Pts',(-16.9962984566318,-20.8339050156273,
-16.7383141359331));
#59857=CARTESIAN_POINT('Ctrl Pts',(-17.061292516445,-20.8918985349615,-16.742630298672));
#59858=CARTESIAN_POINT('Ctrl Pts',(-17.1290155886979,-20.9463984154319,
-16.7469464614109));
#59859=CARTESIAN_POINT('Ctrl Pts',(-17.1945325889952,-20.9991229680282,
-16.7511220256026));
#59860=CARTESIAN_POINT('Ctrl Pts',(-17.2626031281003,-21.0485777582944,
-16.7552975897943));
#59861=CARTESIAN_POINT('Ctrl Pts',(-17.3328600861971,-21.0945234985756,
-16.759473153986));
#59862=CARTESIAN_POINT('Ctrl Pts',(-17.4066655562275,-21.1427898489728,
-16.7638596159985));
#59863=CARTESIAN_POINT('Ctrl Pts',(-17.4828836173808,-21.1871830552703,
-16.7682460780111));
#59864=CARTESIAN_POINT('Ctrl Pts',(-17.5610602937788,-21.2274807064816,
-16.7726325400236));
#59865=CARTESIAN_POINT('Ctrl Pts',(-17.6392369701769,-21.2677783576928,
-16.7770190020362));
#59866=CARTESIAN_POINT('Ctrl Pts',(-17.719371701741,-21.3039802842616,-16.7814054640487));
#59867=CARTESIAN_POINT('Ctrl Pts',(-17.8009895271371,-21.3359235427186,
-16.7857919260613));
#59868=CARTESIAN_POINT('Ctrl Pts',(-17.8788519954,-21.3663970445028,-16.7899765604543));
#59869=CARTESIAN_POINT('Ctrl Pts',(-17.9583538968788,-21.3931085897472,
-16.7941611948473));
#59870=CARTESIAN_POINT('Ctrl Pts',(-18.0390969463692,-21.4158810332592,
-16.7983458292404));
#59871=CARTESIAN_POINT('Ctrl Pts',(-18.1197250681227,-21.4386210630166,
-16.8025245073243));
#59872=CARTESIAN_POINT('Ctrl Pts',(-18.2015903898501,-21.4574330041517,
-16.8067031854083));
#59873=CARTESIAN_POINT('Ctrl Pts',(-18.2842754534887,-21.4721880549406,
-16.8108818634922));
#59874=CARTESIAN_POINT('Ctrl Pts',(-18.3684425874682,-21.4872075794106,
-16.8151354413777));
#59875=CARTESIAN_POINT('Ctrl Pts',(-18.4534586911853,-21.49802316776,-16.8193890192631));
#59876=CARTESIAN_POINT('Ctrl Pts',(-18.538868095807,-21.5045523579284,-16.8236425971485));
#59877=CARTESIAN_POINT('Ctrl Pts',(-18.6226216724574,-21.5109549670048,
-16.8278137111265));
#59878=CARTESIAN_POINT('Ctrl Pts',(-18.7067529564692,-21.5132358584627,
-16.8319848251044));
#59879=CARTESIAN_POINT('Ctrl Pts',(-18.7908245916082,-21.5113692515517,
-16.8361559390824));
#59880=CARTESIAN_POINT('Ctrl Pts',(-18.8748680156982,-21.5095032709988,
-16.8403256534027));
#59881=CARTESIAN_POINT('Ctrl Pts',(-18.9588513711302,-21.503492566284,-16.8444953677231));
#59882=CARTESIAN_POINT('Ctrl Pts',(-19.0423370360803,-21.4933634671533,
-16.8486650820435));
#59883=CARTESIAN_POINT('Ctrl Pts',(-19.1258197302523,-21.4832347284594,
-16.8528346479875));
#59884=CARTESIAN_POINT('Ctrl Pts',(-19.2088043125731,-21.4689879429832,
-16.8570042139316));
#59885=CARTESIAN_POINT('Ctrl Pts',(-19.2908593851774,-21.4507011876453,
-16.8611737798756));
#59886=CARTESIAN_POINT('Ctrl Pts',(-19.3757994129086,-21.4317714925488,
-16.8654899426145));
#59887=CARTESIAN_POINT('Ctrl Pts',(-19.4597428368621,-21.4085125658604,
-16.8698061053535));
#59888=CARTESIAN_POINT('Ctrl Pts',(-19.5422258260852,-21.381067931131,-16.8741222680924));
#59889=CARTESIAN_POINT('Ctrl Pts',(-19.6220219406102,-21.3545173024912,
-16.8782978322841));
#59890=CARTESIAN_POINT('Ctrl Pts',(-19.7004508845915,-21.3240496914869,
-16.8824733964757));
#59891=CARTESIAN_POINT('Ctrl Pts',(-19.7771127399862,-21.2898442659165,
-16.8866489606674));
#59892=CARTESIAN_POINT('Ctrl Pts',(-19.8576466034505,-21.2539112056161,
-16.8910354226799));
#59893=CARTESIAN_POINT('Ctrl Pts',(-19.9362296554817,-21.2138530785412,
-16.8954218846925));
#59894=CARTESIAN_POINT('Ctrl Pts',(-20.0124291551049,-21.169931219713,-16.899808346705));
#59895=CARTESIAN_POINT('Ctrl Pts',(-20.0886286547281,-21.1260093608849,
-16.9041948087175));
#59896=CARTESIAN_POINT('Ctrl Pts',(-20.1624441562134,-21.0782241494638,
-16.9085812707301));
#59897=CARTESIAN_POINT('Ctrl Pts',(-20.2334815623277,-21.0268867545577,
-16.9129677327426));
#59898=CARTESIAN_POINT('Ctrl Pts',(-20.3007008312569,-20.9783086554537,
-16.9171184300413));
#59899=CARTESIAN_POINT('Ctrl Pts',(-20.3656920487852,-20.9263629083339,
-16.9212691273401));
#59900=CARTESIAN_POINT('Ctrl Pts',(-20.4280939407346,-20.8712826055499,
-16.9254198246388));
#59901=CARTESIAN_POINT('Ctrl Pts',(-20.4904067758306,-20.816280910614,-16.9295645982704));
#59902=CARTESIAN_POINT('Ctrl Pts',(-20.5501372744547,-20.758153849065,-16.9337093719019));
#59903=CARTESIAN_POINT('Ctrl Pts',(-20.6069541187602,-20.6971770308536,
-16.9378541455334));
#59904=CARTESIAN_POINT('Ctrl Pts',(-20.6637057912846,-20.636270156123,-16.9419941649009));
#59905=CARTESIAN_POINT('Ctrl Pts',(-20.7175501324576,-20.5725203603438,
-16.9461341842684));
#59906=CARTESIAN_POINT('Ctrl Pts',(-20.7681909845743,-20.5062416280221,
-16.9502742036359));
#59907=CARTESIAN_POINT('Ctrl Pts',(-20.8188004163148,-20.4400040186795,
-16.9544116543072));
#59908=CARTESIAN_POINT('Ctrl Pts',(-20.8662100198436,-20.3712409577298,
-16.9585491049784));
#59909=CARTESIAN_POINT('Ctrl Pts',(-20.9101632231194,-20.3003002730633,
-16.9626865556497));
#59910=CARTESIAN_POINT('Ctrl Pts',(-20.9541028768145,-20.2293814574863,
-16.9668227308571));
#59911=CARTESIAN_POINT('Ctrl Pts',(-20.9945879994369,-20.1562867489274,
-16.9709589060645));
#59912=CARTESIAN_POINT('Ctrl Pts',(-21.0314055962389,-20.0813925475095,
-16.9750950812719));
#59913=CARTESIAN_POINT('Ctrl Pts',(-21.0682233367814,-20.0064980536955,
-16.9792312726275));
#59914=CARTESIAN_POINT('Ctrl Pts',(-21.101373318238,-19.9298044742117,-16.983367463983));
#59915=CARTESIAN_POINT('Ctrl Pts',(-21.1306893947114,-19.8517110343203,
-16.9875036553386));
#59916=CARTESIAN_POINT('Ctrl Pts',(-21.1600333335746,-19.773543373383,-16.9916437777855));
#59917=CARTESIAN_POINT('Ctrl Pts',(-21.1855359272153,-19.6939736349119,
-16.9957839002324));
#59918=CARTESIAN_POINT('Ctrl Pts',(-21.2070801670876,-19.6134185415892,
-16.9999240226793));
#59919=CARTESIAN_POINT('Ctrl Pts',(-21.2286351815299,-19.5328231615589,
-17.0040662156583));
#59920=CARTESIAN_POINT('Ctrl Pts',(-21.2462278030767,-19.4512419037244,
-17.0082084086373));
#59921=CARTESIAN_POINT('Ctrl Pts',(-21.2597921942375,-19.3691016561091,
-17.0123506016163));
#59922=CARTESIAN_POINT('Ctrl Pts',(-21.2733789861849,-19.286825758752,-17.016499635181));
#59923=CARTESIAN_POINT('Ctrl Pts',(-21.2829242114339,-19.2039894937101,
-17.0206486687457));
#59924=CARTESIAN_POINT('Ctrl Pts',(-21.2884139728529,-19.1210244221818,
-17.0247977023105));
#59925=CARTESIAN_POINT('Ctrl Pts',(-21.2921595270972,-19.0644190158498,
-17.0276285047975));
#59926=CARTESIAN_POINT('Ctrl Pts',(-21.2940183320645,-19.0077536994293,
-17.0304593072845));
#59927=CARTESIAN_POINT('Ctrl Pts',(-21.2939998636668,-18.9511645205579,
-17.0332901097715));
#59928=CARTESIAN_POINT('Ctrl Pts',(-21.2979001731334,-18.9511632476561,
-17.0332901097715));
#59929=CARTESIAN_POINT('Ctrl Pts',(-21.2980948808476,-18.9054257555603,
-17.0355745863224));
#59930=CARTESIAN_POINT('Ctrl Pts',(-21.2762380388006,-18.0111494605167,
-17.0802509984337));
#59931=CARTESIAN_POINT('Ctrl Pts',(-20.2331955662249,-16.3222274596702,
-17.1673193461055));
#59932=CARTESIAN_POINT('Ctrl Pts',(-18.131091639517,-16.2828821145566,-17.2595383994549));
#59933=CARTESIAN_POINT('Ctrl Pts',(-17.2909884432664,-16.8286169939874,
-17.3093655172438));
#59934=CARTESIAN_POINT('Ctrl Pts',(-17.1735447326512,-16.9206895600706,
-17.3168006994722));
#59935=CARTESIAN_POINT('',(-21.2938494935628,-18.9531967451209,-16.9667098397524));
#59936=CARTESIAN_POINT('Ctrl Pts',(-21.290325207156,-18.9531940791588,-16.9667098902285));
#59937=CARTESIAN_POINT('Ctrl Pts',(-21.2882101978943,-18.4498774972589,
-16.9916592919231));
#59938=CARTESIAN_POINT('Ctrl Pts',(-20.9008594754591,-17.088363994255,-17.0590006291781));
#59939=CARTESIAN_POINT('Ctrl Pts',(-18.9946005776491,-16.0873964875648,
-17.1534395121067));
#59940=CARTESIAN_POINT('Ctrl Pts',(-17.611718042421,-16.5944337234933,-17.2229289933409));
#59941=CARTESIAN_POINT('Ctrl Pts',(-17.1762220723153,-16.9241895431828,
-17.2500265390144));
#59942=CARTESIAN_POINT('Ctrl Pts',(-17.1744641548914,-16.9218650419685,
-16.4501666890971));
#59943=CARTESIAN_POINT('Ctrl Pts',(-17.1078206357512,-16.9730601393841,
-16.4543369048848));
#59944=CARTESIAN_POINT('Ctrl Pts',(-17.0436639638458,-17.0275684362512,
-16.4585071206726));
#59945=CARTESIAN_POINT('Ctrl Pts',(-16.9823340376993,-17.0851131912949,
-16.4626773364604));
#59946=CARTESIAN_POINT('Ctrl Pts',(-16.9210149346286,-17.1426477912433,
-16.4668468163177));
#59947=CARTESIAN_POINT('Ctrl Pts',(-16.86252192151,-17.2032174699326,-16.471016296175));
#59948=CARTESIAN_POINT('Ctrl Pts',(-16.8071597460482,-17.2665070051314,
-16.4751857760323));
#59949=CARTESIAN_POINT('Ctrl Pts',(-16.7517907333809,-17.3298043565614,
-16.4793557708186));
#59950=CARTESIAN_POINT('Ctrl Pts',(-16.6995536280125,-17.395821884368,-16.483525765605));
#59951=CARTESIAN_POINT('Ctrl Pts',(-16.6507135127919,-17.4642105618684,
-16.4876957603913));
#59952=CARTESIAN_POINT('Ctrl Pts',(-16.601820905061,-17.5326727423353,-16.4918702370158));
#59953=CARTESIAN_POINT('Ctrl Pts',(-16.5563328438427,-17.6035107849438,
-16.4960447136403));
#59954=CARTESIAN_POINT('Ctrl Pts',(-16.5144712872111,-17.6763463271305,
-16.5002191902648));
#59955=CARTESIAN_POINT('Ctrl Pts',(-16.4725853040748,-17.7492243693543,
-16.504396102725));
#59956=CARTESIAN_POINT('Ctrl Pts',(-16.4343302474926,-17.8241018219044,
-16.5085730151852));
#59957=CARTESIAN_POINT('Ctrl Pts',(-16.3998811614755,-17.9005775122982,
-16.5127499276454));
#59958=CARTESIAN_POINT('Ctrl Pts',(-16.3653738366734,-17.9771824906297,
-16.516933901492));
#59959=CARTESIAN_POINT('Ctrl Pts',(-16.334685497607,-18.0553906735663,-16.5211178753385));
#59960=CARTESIAN_POINT('Ctrl Pts',(-16.3079421752585,-18.1347831187435,
-16.5253018491851));
#59961=CARTESIAN_POINT('Ctrl Pts',(-16.2918495927868,-18.182556894006,-16.5278195223189));
#59962=CARTESIAN_POINT('Ctrl Pts',(-16.2771845020012,-18.2307592098647,
-16.5303371954527));
#59963=CARTESIAN_POINT('Ctrl Pts',(-16.2639654295305,-18.2792970784325,
-16.5328548685865));
#59964=CARTESIAN_POINT('Ctrl Pts',(-16.2419939573157,-18.3599720602031,
-16.5370395029795));
#59965=CARTESIAN_POINT('Ctrl Pts',(-16.223938199736,-18.4418747378536,-16.5412241373726));
#59966=CARTESIAN_POINT('Ctrl Pts',(-16.2099316900943,-18.5245901651461,
-16.5454087717656));
#59967=CARTESIAN_POINT('Ctrl Pts',(-16.1959451169854,-18.6071878572661,
-16.5495874498496));
#59968=CARTESIAN_POINT('Ctrl Pts',(-16.1859964196337,-18.6905955514665,
-16.5537661279335));
#59969=CARTESIAN_POINT('Ctrl Pts',(-16.18016901464,-18.7743844088627,-16.5579448060175));
#59970=CARTESIAN_POINT('Ctrl Pts',(-16.1742371575999,-18.8596751213096,
-16.5621983839029));
#59971=CARTESIAN_POINT('Ctrl Pts',(-16.1725759211884,-18.9453603308628,
-16.5664519617884));
#59972=CARTESIAN_POINT('Ctrl Pts',(-16.1752185615464,-19.0309781629659,
-16.5707055396738));
#59973=CARTESIAN_POINT('Ctrl Pts',(-16.1778099691644,-19.1149361263243,
-16.5748766536517));
#59974=CARTESIAN_POINT('Ctrl Pts',(-16.1845398497979,-19.1988288204161,
-16.5790477676297));
#59975=CARTESIAN_POINT('Ctrl Pts',(-16.1953870618678,-19.2822186402182,
-16.5832188816076));
#59976=CARTESIAN_POINT('Ctrl Pts',(-16.2062306340508,-19.3655804777609,
-16.587388595928));
#59977=CARTESIAN_POINT('Ctrl Pts',(-16.2211887344791,-19.4484393203328,
-16.5915583102484));
#59978=CARTESIAN_POINT('Ctrl Pts',(-16.2401883815476,-19.5303628719688,
-16.5957280245688));
#59979=CARTESIAN_POINT('Ctrl Pts',(-16.2591873525272,-19.6122835084131,
-16.5998975905128));
#59980=CARTESIAN_POINT('Ctrl Pts',(-16.2822274794425,-19.6932684721477,
-16.6040671564568));
#59981=CARTESIAN_POINT('Ctrl Pts',(-16.3091849959465,-19.7728971897364,
-16.6082367224009));
#59982=CARTESIAN_POINT('Ctrl Pts',(-16.3370903054751,-19.8553255548029,
-16.6125528851398));
#59983=CARTESIAN_POINT('Ctrl Pts',(-16.3691934316989,-19.9363000284499,
-16.6168690478787));
#59984=CARTESIAN_POINT('Ctrl Pts',(-16.4053020683427,-20.015374789571,-16.6211852106176));
#59985=CARTESIAN_POINT('Ctrl Pts',(-16.4402344699458,-20.0918736986657,
-16.6253607748093));
#59986=CARTESIAN_POINT('Ctrl Pts',(-16.4789151719815,-20.1665943642433,
-16.629536339001));
#59987=CARTESIAN_POINT('Ctrl Pts',(-16.5211232637328,-20.2391583236289,
-16.6337119031927));
#59988=CARTESIAN_POINT('Ctrl Pts',(-16.5654631858582,-20.3153873160987,
-16.6380983652052));
#59989=CARTESIAN_POINT('Ctrl Pts',(-16.6136958800291,-20.3892355173248,
-16.6424848272177));
#59990=CARTESIAN_POINT('Ctrl Pts',(-16.6655152292138,-20.460300617591,-16.6468712892303));
#59991=CARTESIAN_POINT('Ctrl Pts',(-16.7173345783985,-20.5313657178572,
-16.6512577512428));
#59992=CARTESIAN_POINT('Ctrl Pts',(-16.7727401579416,-20.5996473145404,
-16.6556442132554));
#59993=CARTESIAN_POINT('Ctrl Pts',(-16.8313804354228,-20.664786849695,-16.6600306752679));
#59994=CARTESIAN_POINT('Ctrl Pts',(-16.8873225868114,-20.7269292182772,
-16.664215309661));
#59995=CARTESIAN_POINT('Ctrl Pts',(-16.9464165382123,-20.7864436190212,
-16.668399944054));
#59996=CARTESIAN_POINT('Ctrl Pts',(-17.0083856645506,-20.842993169023,-16.6725845784471));
#59997=CARTESIAN_POINT('Ctrl Pts',(-17.0702665855077,-20.8994622277397,
-16.676763256531));
#59998=CARTESIAN_POINT('Ctrl Pts',(-17.1350142155918,-20.9529745107155,
-16.6809419346149));
#59999=CARTESIAN_POINT('Ctrl Pts',(-17.2023131209901,-21.0032277554355,
-16.6851206126989));
#60000=CARTESIAN_POINT('Ctrl Pts',(-17.2708183109008,-21.0543817534507,
-16.6893741905843));
#60001=CARTESIAN_POINT('Ctrl Pts',(-17.3419668163949,-21.102158369159,-16.6936277684697));
#60002=CARTESIAN_POINT('Ctrl Pts',(-17.4153882749822,-21.1462796354716,
-16.6978813463552));
#60003=CARTESIAN_POINT('Ctrl Pts',(-17.4873863153245,-21.1895455249412,
-16.7020524603331));
#60004=CARTESIAN_POINT('Ctrl Pts',(-17.5615695514937,-21.2292962845163,
-16.7062235743111));
#60005=CARTESIAN_POINT('Ctrl Pts',(-17.637558583382,-21.26531282362,-16.710394688289));
#60006=CARTESIAN_POINT('Ctrl Pts',(-17.7135221164167,-21.3013172770261,
-16.7145644026094));
#60007=CARTESIAN_POINT('Ctrl Pts',(-17.7912898263826,-21.3335898016786,
-16.7187341169298));
#60008=CARTESIAN_POINT('Ctrl Pts',(-17.8704587172267,-21.3619577699508,
-16.7229038312502));
#60009=CARTESIAN_POINT('Ctrl Pts',(-17.9496247909019,-21.3903247287689,
-16.7270733971942));
#60010=CARTESIAN_POINT('Ctrl Pts',(-18.030191512963,-21.4147872530805,-16.7312429631382));
#60011=CARTESIAN_POINT('Ctrl Pts',(-18.1117382553313,-21.4352217623728,
-16.7354125290823));
#60012=CARTESIAN_POINT('Ctrl Pts',(-18.1961520805624,-21.4563747238031,
-16.7397286918212));
#60013=CARTESIAN_POINT('Ctrl Pts',(-18.2816156117522,-21.4732110218616,
-16.7440448545601));
#60014=CARTESIAN_POINT('Ctrl Pts',(-18.3676498921637,-21.4856510411831,
-16.748361017299));
#60015=CARTESIAN_POINT('Ctrl Pts',(-18.4508816149399,-21.4976858281837,
-16.7525365814907));
#60016=CARTESIAN_POINT('Ctrl Pts',(-18.5346470002632,-21.5056063582132,
-16.7567121456824));
#60017=CARTESIAN_POINT('Ctrl Pts',(-18.6185082461362,-21.5093935275568,
-16.7608877098741));
#60018=CARTESIAN_POINT('Ctrl Pts',(-18.7066051241771,-21.5133719778208,
-16.7652741718866));
#60019=CARTESIAN_POINT('Ctrl Pts',(-18.7948072172264,-21.5127885456943,
-16.7696606338992));
#60020=CARTESIAN_POINT('Ctrl Pts',(-18.8826105511363,-21.5076828645376,
-16.7740470959117));
#60021=CARTESIAN_POINT('Ctrl Pts',(-18.9704138850463,-21.5025771833809,
-16.7784335579242));
#60022=CARTESIAN_POINT('Ctrl Pts',(-19.0578178914167,-21.4929493923299,
-16.7828200199368));
#60023=CARTESIAN_POINT('Ctrl Pts',(-19.1443308019265,-21.4789009939035,
-16.7872064819493));
#60024=CARTESIAN_POINT('Ctrl Pts',(-19.226863125181,-21.4654989831134,-16.7913911163424));
#60025=CARTESIAN_POINT('Ctrl Pts',(-19.3088917529366,-21.4480243381486,
-16.7955757507354));
#60026=CARTESIAN_POINT('Ctrl Pts',(-19.3899836880773,-21.4265273085938,
-16.7997603851285));
#60027=CARTESIAN_POINT('Ctrl Pts',(-19.4709601988853,-21.4050608773999,
-16.8039390632124));
#60028=CARTESIAN_POINT('Ctrl Pts',(-19.5510022244941,-21.3795835508679,
-16.8081177412964));
#60029=CARTESIAN_POINT('Ctrl Pts',(-19.6296848716226,-21.3501969499494,
-16.8122964193803));
#60030=CARTESIAN_POINT('Ctrl Pts',(-19.7097778486527,-21.3202836153291,
-16.8165499972657));
#60031=CARTESIAN_POINT('Ctrl Pts',(-19.7884617582359,-21.2863195576314,
-16.8208035751512));
#60032=CARTESIAN_POINT('Ctrl Pts',(-19.8653024038482,-21.2484657347862,
-16.8250571530366));
#60033=CARTESIAN_POINT('Ctrl Pts',(-19.9406533436032,-21.2113457821626,
-16.8292282670146));
#60034=CARTESIAN_POINT('Ctrl Pts',(-20.0142314204538,-21.1704857525211,
-16.8333993809925));
#60035=CARTESIAN_POINT('Ctrl Pts',(-20.0856470518143,-21.1260860717372,
-16.8375704949705));
#60036=CARTESIAN_POINT('Ctrl Pts',(-20.15703871897,-21.081701289695,-16.8417402092909));
#60037=CARTESIAN_POINT('Ctrl Pts',(-20.2262689913883,-21.0337794581181,
-16.8459099236112));
#60038=CARTESIAN_POINT('Ctrl Pts',(-20.2929745824341,-20.9825659928514,
-16.8500796379316));
#60039=CARTESIAN_POINT('Ctrl Pts',(-20.3596777998085,-20.9313543499797,
-16.8542492038756));
#60040=CARTESIAN_POINT('Ctrl Pts',(-20.4238561500589,-20.8768515871279,
-16.8584187698197));
#60041=CARTESIAN_POINT('Ctrl Pts',(-20.4851780435301,-20.8193444941569,
-16.8625883357637));
#60042=CARTESIAN_POINT('Ctrl Pts',(-20.5486559391271,-20.7598155227396,
-16.8669044985026));
#60043=CARTESIAN_POINT('Ctrl Pts',(-20.6090723898813,-20.6970673867193,
-16.8712206612416));
#60044=CARTESIAN_POINT('Ctrl Pts',(-20.6661012016726,-20.6314597186284,
-16.8755368239805));
#60045=CARTESIAN_POINT('Ctrl Pts',(-20.7212723059182,-20.5679892134248,
-16.8797123881722));
#60046=CARTESIAN_POINT('Ctrl Pts',(-20.7732728325614,-20.5018430132075,
-16.8838879523639));
#60047=CARTESIAN_POINT('Ctrl Pts',(-20.8218497444836,-20.4333788996943,
-16.8880635165556));
#60048=CARTESIAN_POINT('Ctrl Pts',(-20.8728801607463,-20.3614568265658,
-16.8924499785681));
#60049=CARTESIAN_POINT('Ctrl Pts',(-20.9201317067406,-20.2869770238507,
-16.8968364405806));
#60050=CARTESIAN_POINT('Ctrl Pts',(-20.9633649162028,-20.2103847068381,
-16.9012229025932));
#60051=CARTESIAN_POINT('Ctrl Pts',(-21.0065981256651,-20.1337923898255,
-16.9056093646057));
#60052=CARTESIAN_POINT('Ctrl Pts',(-21.0458128079223,-20.0550881117615,
-16.9099958266183));
#60053=CARTESIAN_POINT('Ctrl Pts',(-21.0808281256648,-19.9747403133684,
-16.9143822886308));
#60054=CARTESIAN_POINT('Ctrl Pts',(-21.1176528956138,-19.890240460661,-16.9189954255354));
#60055=CARTESIAN_POINT('Ctrl Pts',(-21.1499518315865,-19.8036540013275,
-16.9236085624399));
#60056=CARTESIAN_POINT('Ctrl Pts',(-21.1775079602931,-19.7154584782318,
-16.9282216993445));
#60057=CARTESIAN_POINT('Ctrl Pts',(-21.2049852187145,-19.6275153855896,
-16.9328216326736));
#60058=CARTESIAN_POINT('Ctrl Pts',(-21.2277466226989,-19.5379726851093,
-16.9374215660027));
#60059=CARTESIAN_POINT('Ctrl Pts',(-21.2456232056933,-19.4473270360306,
-16.9420214993319));
#60060=CARTESIAN_POINT('Ctrl Pts',(-21.2634117418665,-19.3571278403517,
-16.9465987767929));
#60061=CARTESIAN_POINT('Ctrl Pts',(-21.2763633328304,-19.2658368103367,
-16.9511760542538));
#60062=CARTESIAN_POINT('Ctrl Pts',(-21.2843593339855,-19.1739623111095,
-16.9557533317148));
#60063=CARTESIAN_POINT('Ctrl Pts',(-21.2907392715843,-19.1006564722762,
-16.9594055003435));
#60064=CARTESIAN_POINT('Ctrl Pts',(-21.2939652250916,-19.0269796001108,
-16.9630576689721));
#60065=CARTESIAN_POINT('Ctrl Pts',(-21.2939997202205,-18.9531968587605,
-16.9667098376008));
#60066=CARTESIAN_POINT('Origin',(-18.734,-18.952,1.76670989022851));
#60067=CARTESIAN_POINT('',(-17.1721129765924,-16.9188350422745,-15.6501589808892));
#60068=CARTESIAN_POINT('',(-17.1744641548914,-16.9218650419685,-15.7166572062078));
#60069=CARTESIAN_POINT('',(-17.1744641548914,-16.9218650419685,1.76670989022851));
#60070=CARTESIAN_POINT('',(-21.2939992944986,-18.9500994299065,-16.2332901098004));
#60071=CARTESIAN_POINT('Ctrl Pts',(-17.1744641548914,-16.9218650419685,
-15.7166572062078));
#60072=CARTESIAN_POINT('Ctrl Pts',(-17.1055401828173,-16.9748119677931,
-15.7209678950746));
#60073=CARTESIAN_POINT('Ctrl Pts',(-17.0393402583663,-17.0312538502349,
-15.7252785839415));
#60074=CARTESIAN_POINT('Ctrl Pts',(-16.9762229031562,-17.0908660236803,
-15.7295892728083));
#60075=CARTESIAN_POINT('Ctrl Pts',(-16.9150839105399,-17.1486097016275,
-15.7337648466093));
#60076=CARTESIAN_POINT('Ctrl Pts',(-16.8568373862815,-17.2093274875522,
-15.7379404204102));
#60077=CARTESIAN_POINT('Ctrl Pts',(-16.8017702605312,-17.2726881665657,
-15.7421159942111));
#60078=CARTESIAN_POINT('Ctrl Pts',(-16.7440303051251,-17.339124224938,-15.7464942406109));
#60079=CARTESIAN_POINT('Ctrl Pts',(-16.6897865650317,-17.4084657801725,
-15.7508724870107));
#60080=CARTESIAN_POINT('Ctrl Pts',(-16.6393195124585,-17.4802956631466,
-15.7552507334104));
#60081=CARTESIAN_POINT('Ctrl Pts',(-16.5888524598854,-17.5521255461208,
-15.7596289798102));
#60082=CARTESIAN_POINT('Ctrl Pts',(-16.5421623367065,-17.6264432299862,
-15.76400722621));
#60083=CARTESIAN_POINT('Ctrl Pts',(-16.4994739740979,-17.7028028820213,
-15.7683854726097));
#60084=CARTESIAN_POINT('Ctrl Pts',(-16.458673348906,-17.7757858064552,-15.7725701070028));
#60085=CARTESIAN_POINT('Ctrl Pts',(-16.4213761508428,-17.8509055642072,
-15.7767547413958));
#60086=CARTESIAN_POINT('Ctrl Pts',(-16.3878121523981,-17.9277917283261,
-15.7809393757889));
#60087=CARTESIAN_POINT('Ctrl Pts',(-16.3542959281507,-18.0045684545072,
-15.7851180538728));
#60088=CARTESIAN_POINT('Ctrl Pts',(-16.3245025312235,-18.0831061749373,
-15.7892967319568));
#60089=CARTESIAN_POINT('Ctrl Pts',(-16.2986164546583,-18.163008880228,-15.7934754100407));
#60090=CARTESIAN_POINT('Ctrl Pts',(-16.2722663887748,-18.2443437840859,
-15.7977289879262));
#60091=CARTESIAN_POINT('Ctrl Pts',(-16.2499653337518,-18.3270926679903,
-15.8019825658116));
#60092=CARTESIAN_POINT('Ctrl Pts',(-16.2318570828657,-18.4108153529206,
-15.806236143697));
#60093=CARTESIAN_POINT('Ctrl Pts',(-16.2140998957582,-18.4929149102322,
-15.810407257675));
#60094=CARTESIAN_POINT('Ctrl Pts',(-16.2003744938965,-18.5759503771067,
-15.8145783716529));
#60095=CARTESIAN_POINT('Ctrl Pts',(-16.1907660223745,-18.6594919914754,
-15.8187494856309));
#60096=CARTESIAN_POINT('Ctrl Pts',(-16.1811607750679,-18.7430055726484,
-15.8229191999512));
#60097=CARTESIAN_POINT('Ctrl Pts',(-16.1756697669882,-18.8270245073658,
-15.8270889142716));
#60098=CARTESIAN_POINT('Ctrl Pts',(-16.1743265551335,-18.9111116685931,
-15.831258628592));
#60099=CARTESIAN_POINT('Ctrl Pts',(-16.172983391076,-18.9951958376385,-15.835428194536));
#60100=CARTESIAN_POINT('Ctrl Pts',(-16.1757877362795,-19.079347768379,-15.8395977604801));
#60101=CARTESIAN_POINT('Ctrl Pts',(-16.182721035153,-19.1631294473286,-15.8437673264241));
#60102=CARTESIAN_POINT('Ctrl Pts',(-16.1898981002617,-19.2498567867541,
-15.848083489163));
#60103=CARTESIAN_POINT('Ctrl Pts',(-16.2014998257647,-19.3361868282292,
-15.8523996519019));
#60104=CARTESIAN_POINT('Ctrl Pts',(-16.2174472402025,-19.4216405084271,
-15.8567158146408));
#60105=CARTESIAN_POINT('Ctrl Pts',(-16.2328751692924,-19.5043105439808,
-15.8608913788325));
#60106=CARTESIAN_POINT('Ctrl Pts',(-16.2523698584565,-19.5861599891147,
-15.8650669430242));
#60107=CARTESIAN_POINT('Ctrl Pts',(-16.2758083142181,-19.6667682393286,
-15.8692425072159));
#60108=CARTESIAN_POINT('Ctrl Pts',(-16.3004305906605,-19.7514478206325,
-15.8736289692284));
#60109=CARTESIAN_POINT('Ctrl Pts',(-16.3294053113242,-19.8347569748338,
-15.8780154312409));
#60110=CARTESIAN_POINT('Ctrl Pts',(-16.3625325554082,-19.9162313826263,
-15.8824018932535));
#60111=CARTESIAN_POINT('Ctrl Pts',(-16.3956597994923,-19.9977057904188,
-15.886788355266));
#60112=CARTESIAN_POINT('Ctrl Pts',(-16.4329392521204,-20.0773449585575,
-15.8911748172785));
#60113=CARTESIAN_POINT('Ctrl Pts',(-16.4741163568262,-20.1547160593073,
-15.8955612792911));
#60114=CARTESIAN_POINT('Ctrl Pts',(-16.5133988419055,-20.2285272010201,
-15.8997459136841));
#60115=CARTESIAN_POINT('Ctrl Pts',(-16.5563744043011,-20.3005491422939,
-15.9039305480772));
#60116=CARTESIAN_POINT('Ctrl Pts',(-16.6028559450592,-20.370388175744,-15.9081151824702));
#60117=CARTESIAN_POINT('Ctrl Pts',(-16.6492713250974,-20.4401278019745,
-15.9122938605541));
#60118=CARTESIAN_POINT('Ctrl Pts',(-16.699182518435,-20.5076903123662,-15.9164725386381));
#60119=CARTESIAN_POINT('Ctrl Pts',(-16.7523564064307,-20.5727062250963,
-15.920651216722));
#60120=CARTESIAN_POINT('Ctrl Pts',(-16.8064833981534,-20.6388875013359,
-15.9249047946075));
#60121=CARTESIAN_POINT('Ctrl Pts',(-16.8639909761113,-20.7024295607927,
-15.9291583724929));
#60122=CARTESIAN_POINT('Ctrl Pts',(-16.924586851981,-20.7629732355217,-15.9334119503784));
#60123=CARTESIAN_POINT('Ctrl Pts',(-16.9840079585538,-20.8223431529748,
-15.9375830643563));
#60124=CARTESIAN_POINT('Ctrl Pts',(-17.0463983458427,-20.8788295671755,
-15.9417541783343));
#60125=CARTESIAN_POINT('Ctrl Pts',(-17.1114427393838,-20.9321282625178,
-15.9459252923122));
#60126=CARTESIAN_POINT('Ctrl Pts',(-17.1764653066504,-20.985409072968,-15.9500950066326));
#60127=CARTESIAN_POINT('Ctrl Pts',(-17.2441397559347,-21.0355039976096,
-15.954264720953));
#60128=CARTESIAN_POINT('Ctrl Pts',(-17.3141166963442,-21.0821482117448,
-15.9584344352733));
#60129=CARTESIAN_POINT('Ctrl Pts',(-17.384091146674,-21.1287907660788,-15.9626040012174));
#60130=CARTESIAN_POINT('Ctrl Pts',(-17.456367541965,-21.1719825996022,-15.9667735671614));
#60131=CARTESIAN_POINT('Ctrl Pts',(-17.5305675384034,-21.2115022262382,
-15.9709431331055));
#60132=CARTESIAN_POINT('Ctrl Pts',(-17.6073763151809,-21.2524113141941,
-15.9752592958444));
#60133=CARTESIAN_POINT('Ctrl Pts',(-17.686246012007,-21.2893849131308,-15.9795754585833));
#60134=CARTESIAN_POINT('Ctrl Pts',(-17.766731066684,-21.3222301176556,-15.9838916213223));
#60135=CARTESIAN_POINT('Ctrl Pts',(-17.8445943291705,-21.3540053930978,
-15.9880671855139));
#60136=CARTESIAN_POINT('Ctrl Pts',(-17.9239688650711,-21.3819169968657,
-15.9922427497056));
#60137=CARTESIAN_POINT('Ctrl Pts',(-18.004434438527,-21.4058406817706,-15.9964183138973));
#60138=CARTESIAN_POINT('Ctrl Pts',(-18.0889641368095,-21.430972695127,-16.0008047759098));
#60139=CARTESIAN_POINT('Ctrl Pts',(-18.1746974182798,-21.451703205484,-16.0051912379224));
#60140=CARTESIAN_POINT('Ctrl Pts',(-18.2611356505439,-21.4679489873631,
-16.0095776999349));
#60141=CARTESIAN_POINT('Ctrl Pts',(-18.3475738828079,-21.4841947692422,
-16.0139641619475));
#60142=CARTESIAN_POINT('Ctrl Pts',(-18.4347164806881,-21.4959558204205,
-16.01835062396));
#60143=CARTESIAN_POINT('Ctrl Pts',(-18.5220617179685,-21.5032119011579,
-16.0227370859726));
#60144=CARTESIAN_POINT('Ctrl Pts',(-18.605388071405,-21.5101341188644,-16.0269217203656));
#60145=CARTESIAN_POINT('Ctrl Pts',(-18.6892089831259,-21.5129825827272,
-16.0311063547587));
#60146=CARTESIAN_POINT('Ctrl Pts',(-18.7730921344112,-21.5117015070174,
-16.0352909891517));
#60147=CARTESIAN_POINT('Ctrl Pts',(-18.8568558884131,-21.5104222547604,
-16.0394696672357));
#60148=CARTESIAN_POINT('Ctrl Pts',(-18.9406812499662,-21.5050251452316,
-16.0436483453196));
#60149=CARTESIAN_POINT('Ctrl Pts',(-19.0241313606303,-21.4955062008139,
-16.0478270234035));
#60150=CARTESIAN_POINT('Ctrl Pts',(-19.1090772545536,-21.4858166361586,
-16.052080601289));
#60151=CARTESIAN_POINT('Ctrl Pts',(-19.1936338320389,-21.471855975481,-16.0563341791744));
#60152=CARTESIAN_POINT('Ctrl Pts',(-19.2773408795583,-21.453675576209,-16.0605877570599));
#60153=CARTESIAN_POINT('Ctrl Pts',(-19.3594251026208,-21.4358476394531,
-16.0647588710378));
#60154=CARTESIAN_POINT('Ctrl Pts',(-19.440691971107,-21.4139622218932,-16.0689299850158));
#60155=CARTESIAN_POINT('Ctrl Pts',(-19.5207150357478,-21.3881197533226,
-16.0731010989937));
#60156=CARTESIAN_POINT('Ctrl Pts',(-19.6007112478764,-21.3622859564419,
-16.0772708133141));
#60157=CARTESIAN_POINT('Ctrl Pts',(-19.6794640476564,-21.3324978868906,
-16.0814405276345));
#60158=CARTESIAN_POINT('Ctrl Pts',(-19.7565616407632,-21.298905982531,-16.0856102419548));
#60159=CARTESIAN_POINT('Ctrl Pts',(-19.8336564904068,-21.2653152735155,
-16.0897798078989));
#60160=CARTESIAN_POINT('Ctrl Pts',(-19.9090958290848,-21.2279211833516,
-16.0939493738429));
#60161=CARTESIAN_POINT('Ctrl Pts',(-19.9824886317269,-21.1869219531001,
-16.098118939787));
#60162=CARTESIAN_POINT('Ctrl Pts',(-20.0584618347702,-21.1444812404909,
-16.1024351025259));
#60163=CARTESIAN_POINT('Ctrl Pts',(-20.1322414512869,-21.098177414705,-16.1067512652648));
#60164=CARTESIAN_POINT('Ctrl Pts',(-20.2034241040028,-21.0482807070084,
-16.1110674280037));
#60165=CARTESIAN_POINT('Ctrl Pts',(-20.2722879892936,-21.0000093793168,
-16.1152429921954));
#60166=CARTESIAN_POINT('Ctrl Pts',(-20.3387211617813,-20.9483759776511,
-16.1194185563871));
#60167=CARTESIAN_POINT('Ctrl Pts',(-20.4023916835426,-20.8936666012181,
-16.1235941205788));
#60168=CARTESIAN_POINT('Ctrl Pts',(-20.4692780519956,-20.8361939842408,
-16.1279805825913));
#60169=CARTESIAN_POINT('Ctrl Pts',(-20.533114929731,-20.7753268941813,-16.1323670446039));
#60170=CARTESIAN_POINT('Ctrl Pts',(-20.5935624370343,-20.7114395535997,
-16.1367535066164));
#60171=CARTESIAN_POINT('Ctrl Pts',(-20.6540099443376,-20.6475522130181,
-16.141139968629));
#60172=CARTESIAN_POINT('Ctrl Pts',(-20.7110677625942,-20.5806451127529,
-16.1455264306415));
#60173=CARTESIAN_POINT('Ctrl Pts',(-20.764447298501,-20.5111291697643,-16.149912892654));
#60174=CARTESIAN_POINT('Ctrl Pts',(-20.8154455601759,-20.4447143500982,
-16.1541036735168));
#60175=CARTESIAN_POINT('Ctrl Pts',(-20.8632791399794,-20.3756679864259,
-16.1582944543796));
#60176=CARTESIAN_POINT('Ctrl Pts',(-20.9076654294935,-20.3043234082959,
-16.1624852352424));
#60177=CARTESIAN_POINT('Ctrl Pts',(-20.9519891627481,-20.233079380358,-16.1666701097864));
#60178=CARTESIAN_POINT('Ctrl Pts',(-20.9928750133147,-20.1595439541276,
-16.1708549843304));
#60179=CARTESIAN_POINT('Ctrl Pts',(-21.0300812471761,-20.0840825528053,
-16.1750398588744));
#60180=CARTESIAN_POINT('Ctrl Pts',(-21.0672460755937,-20.0087051296902,
-16.1792200762261));
#60181=CARTESIAN_POINT('Ctrl Pts',(-21.1007392197538,-19.9314063968234,
-16.1834002935778));
#60182=CARTESIAN_POINT('Ctrl Pts',(-21.1303635397436,-19.8525785836825,
-16.1875805109294));
#60183=CARTESIAN_POINT('Ctrl Pts',(-21.159964013956,-19.7738142221411,-16.1917573634601));
#60184=CARTESIAN_POINT('Ctrl Pts',(-21.1857016914125,-19.6935236530682,
-16.1959342159908));
#60185=CARTESIAN_POINT('Ctrl Pts',(-21.2074270380285,-19.6121202068937,
-16.2001110685216));
#60186=CARTESIAN_POINT('Ctrl Pts',(-21.2291418983467,-19.5307560521882,
-16.2042859049869));
#60187=CARTESIAN_POINT('Ctrl Pts',(-21.2468481598046,-19.4482805298198,
-16.2084607414522));
#60188=CARTESIAN_POINT('Ctrl Pts',(-21.2604461548152,-19.3651220483335,
-16.2126355779175));
#60189=CARTESIAN_POINT('Ctrl Pts',(-21.2740449836494,-19.2819584676034,
-16.216810670382));
#60190=CARTESIAN_POINT('Ctrl Pts',(-21.2835349604933,-19.1981122945302,
-16.2209857628466));
#60191=CARTESIAN_POINT('Ctrl Pts',(-21.2888677421722,-19.1140210480402,
-16.2251608553111));
#60192=CARTESIAN_POINT('Ctrl Pts',(-21.2923288662564,-19.0594434830793,
-16.2278706067979));
#60193=CARTESIAN_POINT('Ctrl Pts',(-21.2940398771788,-19.0047628516758,
-16.2305803582847));
#60194=CARTESIAN_POINT('Ctrl Pts',(-21.293999294499,-18.9500994304893,-16.2332901097715));
#60195=CARTESIAN_POINT('Ctrl Pts',(-21.2939992944986,-18.9500994299065,
-16.2332901098004));
#60196=CARTESIAN_POINT('Ctrl Pts',(-21.2939272486892,-18.8530563258845,
-16.2381006886061));
#60197=CARTESIAN_POINT('Ctrl Pts',(-21.2883332378637,-18.7562381388316,
-16.2429112674119));
#60198=CARTESIAN_POINT('Ctrl Pts',(-21.277317503626,-18.6602191305971,-16.2477218462176));
#60199=CARTESIAN_POINT('Ctrl Pts',(-21.2661096544806,-18.5625255464771,
-16.2526163217373));
#60200=CARTESIAN_POINT('Ctrl Pts',(-21.2492893600035,-18.4656594493969,
-16.2575107972569));
#60201=CARTESIAN_POINT('Ctrl Pts',(-21.2270132516535,-18.3702054253606,
-16.2624052727766));
#60202=CARTESIAN_POINT('Ctrl Pts',(-21.2047371433035,-18.2747514013242,
-16.2672997482962));
#60203=CARTESIAN_POINT('Ctrl Pts',(-21.1770053785921,-18.1807095711097,
-16.2721942238158));
#60204=CARTESIAN_POINT('Ctrl Pts',(-21.1440235064311,-18.088642195582,-16.2770886993355));
#60205=CARTESIAN_POINT('Ctrl Pts',(-21.1158249638011,-18.0099272639074,
-16.2812733337285));
#60206=CARTESIAN_POINT('Ctrl Pts',(-21.0837134704203,-17.9324488089605,
-16.2854579681216));
#60207=CARTESIAN_POINT('Ctrl Pts',(-21.0478172393664,-17.856623451588,-16.2896426025146));
#60208=CARTESIAN_POINT('Ctrl Pts',(-21.0119721021543,-17.7809060222264,
-16.2938212805986));
#60209=CARTESIAN_POINT('Ctrl Pts',(-20.9723531229121,-17.7068374289185,
-16.2979999586825));
#60210=CARTESIAN_POINT('Ctrl Pts',(-20.9291375533229,-17.6348169747558,
-16.3021786367665));
#60211=CARTESIAN_POINT('Ctrl Pts',(-20.8851473757074,-17.5615056057125,
-16.3064322146519));
#60212=CARTESIAN_POINT('Ctrl Pts',(-20.8374305643562,-17.4903169777088,
-16.3106857925373));
#60213=CARTESIAN_POINT('Ctrl Pts',(-20.7862244101174,-17.4216487427658,
-16.3149393704228));
#60214=CARTESIAN_POINT('Ctrl Pts',(-20.7360109870992,-17.3543117755523,
-16.3191104844007));
#60215=CARTESIAN_POINT('Ctrl Pts',(-20.6824425969515,-17.2893987337786,
-16.3232815983787));
#60216=CARTESIAN_POINT('Ctrl Pts',(-20.6257872198942,-17.2272562176819,
-16.3274527123566));
#60217=CARTESIAN_POINT('Ctrl Pts',(-20.5691508540959,-17.1651345541068,
-16.331622426677));
#60218=CARTESIAN_POINT('Ctrl Pts',(-20.5094298683179,-17.105781909528,-16.3357921409974));
#60219=CARTESIAN_POINT('Ctrl Pts',(-20.4469316957118,-17.0495108394984,
-16.3399618553177));
#60220=CARTESIAN_POINT('Ctrl Pts',(-20.3844357470588,-16.993241771835,-16.3441314212618));
#60221=CARTESIAN_POINT('Ctrl Pts',(-20.3191631505139,-16.9400543678782,
-16.3483009872058));
#60222=CARTESIAN_POINT('Ctrl Pts',(-20.2514562536418,-16.890222485746,-16.3524705531499));
#60223=CARTESIAN_POINT('Ctrl Pts',(-20.1813688658012,-16.8386385761122,
-16.3567867158888));
#60224=CARTESIAN_POINT('Ctrl Pts',(-20.108673237446,-16.7906508514966,-16.3611028786277));
#60225=CARTESIAN_POINT('Ctrl Pts',(-20.0337823603675,-16.7465146076935,
-16.3654190413666));
#60226=CARTESIAN_POINT('Ctrl Pts',(-19.9613310457328,-16.7038160973899,
-16.3695946055583));
#60227=CARTESIAN_POINT('Ctrl Pts',(-19.8868257455389,-16.6647221743667,
-16.37377016975));
#60228=CARTESIAN_POINT('Ctrl Pts',(-19.8106643175706,-16.6294165359948,
-16.3779457339417));
#60229=CARTESIAN_POINT('Ctrl Pts',(-19.7306561569322,-16.59232769376,-16.3823321959542));
#60230=CARTESIAN_POINT('Ctrl Pts',(-19.6488207114385,-16.5594201038734,
-16.3867186579667));
#60231=CARTESIAN_POINT('Ctrl Pts',(-19.5656393424726,-16.5308482071436,
-16.3911051199793));
#60232=CARTESIAN_POINT('Ctrl Pts',(-19.4824579735068,-16.5022763104138,
-16.3954915819918));
#60233=CARTESIAN_POINT('Ctrl Pts',(-19.3979312597771,-16.4780401936422,
-16.3998780440044));
#60234=CARTESIAN_POINT('Ctrl Pts',(-19.3125527301389,-16.4582324209244,
-16.4042645060169));
#60235=CARTESIAN_POINT('Ctrl Pts',(-19.2310959760785,-16.4393344980203,
-16.408449480376));
#60236=CARTESIAN_POINT('Ctrl Pts',(-19.1485607218034,-16.424396672901,-16.412634454735));
#60237=CARTESIAN_POINT('Ctrl Pts',(-19.0653667817925,-16.4135366742999,
-16.4168194290941));
#60238=CARTESIAN_POINT('Ctrl Pts',(-18.9823149545929,-16.4026952268689,
-16.4209972546335));
#60239=CARTESIAN_POINT('Ctrl Pts',(-18.8986071312438,-16.3959178140196,
-16.425175080173));
#60240=CARTESIAN_POINT('Ctrl Pts',(-18.8146747411091,-16.39327149034,-16.4293529057124));
#60241=CARTESIAN_POINT('Ctrl Pts',(-18.7308239310132,-16.3906277388162,
-16.4335266705171));
#60242=CARTESIAN_POINT('Ctrl Pts',(-18.6467494445236,-16.3921071193267,
-16.4377004353219));
#60243=CARTESIAN_POINT('Ctrl Pts',(-18.5628884909385,-16.397724985154,-16.4418742001266));
#60244=CARTESIAN_POINT('Ctrl Pts',(-18.4790838891877,-16.403339075958,-16.4460451602971));
#60245=CARTESIAN_POINT('Ctrl Pts',(-18.3954929930032,-16.4130860985613,
-16.4502161204676));
#60246=CARTESIAN_POINT('Ctrl Pts',(-18.3125523070062,-16.4269293391926,
-16.4543870806381));
#60247=CARTESIAN_POINT('Ctrl Pts',(-18.22964247348,-16.4407674303829,-16.458556489285));
#60248=CARTESIAN_POINT('Ctrl Pts',(-18.1473828227084,-16.4586986359206,
-16.462725897932));
#60249=CARTESIAN_POINT('Ctrl Pts',(-18.0662026746028,-16.4806346421073,
-16.4668953065789));
#60250=CARTESIAN_POINT('Ctrl Pts',(-17.9849897282849,-16.5025795108275,
-16.4710663997405));
#60251=CARTESIAN_POINT('Ctrl Pts',(-17.9048576030274,-16.5285323016448,
-16.4752374929021));
#60252=CARTESIAN_POINT('Ctrl Pts',(-17.8262226566495,-16.5583541834892,
-16.4794085860637));
#60253=CARTESIAN_POINT('Ctrl Pts',(-17.7475755658492,-16.5881806710407,
-16.4835803234112));
#60254=CARTESIAN_POINT('Ctrl Pts',(-17.6704265406045,-16.6218772648513,
-16.4877520607586));
#60255=CARTESIAN_POINT('Ctrl Pts',(-17.5951721110539,-16.6592568745368,
-16.491923798106));
#60256=CARTESIAN_POINT('Ctrl Pts',(-17.5198228508105,-16.6966835875531,
-16.496100792403));
#60257=CARTESIAN_POINT('Ctrl Pts',(-17.4463733639788,-16.7378023734028,
-16.5002777867));
#60258=CARTESIAN_POINT('Ctrl Pts',(-17.3751954107008,-16.7823801973388,
-16.504454780997));
#60259=CARTESIAN_POINT('Ctrl Pts',(-17.3060362383624,-16.8256936850985,
-16.508513305514));
#60260=CARTESIAN_POINT('Ctrl Pts',(-17.2390217557067,-16.8722723328004,
-16.5125718300309));
#60261=CARTESIAN_POINT('Ctrl Pts',(-17.1744641548915,-16.9218650419685,
-16.5166303545479));
#60262=CARTESIAN_POINT('',(-21.2939994369002,-18.9536979607663,-16.1667098902285));
#60263=CARTESIAN_POINT('Ctrl Pts',(-21.2939994369002,-18.9536979607663,
-16.1667098902285));
#60264=CARTESIAN_POINT('Ctrl Pts',(-21.2940542005915,-18.8711312597184,
-16.1708335669039));
#60265=CARTESIAN_POINT('Ctrl Pts',(-21.2901102644712,-18.7884072256502,
-16.1749572435793));
#60266=CARTESIAN_POINT('Ctrl Pts',(-21.282148407848,-18.7059518510906,-16.1790809202548));
#60267=CARTESIAN_POINT('Ctrl Pts',(-21.274150019936,-18.6231181475505,-16.1832235175451));
#60268=CARTESIAN_POINT('Ctrl Pts',(-21.2620966823449,-18.5405560554535,
-16.1873661148355));
#60269=CARTESIAN_POINT('Ctrl Pts',(-21.2460219433306,-18.45869912201,-16.1915087121259));
#60270=CARTESIAN_POINT('Ctrl Pts',(-21.2300543085101,-18.3773875921873,
-16.1956237077524));
#60271=CARTESIAN_POINT('Ctrl Pts',(-21.2101187777555,-18.2967723256484,
-16.1997387033789));
#60272=CARTESIAN_POINT('Ctrl Pts',(-21.1863001253011,-18.2172727748014,
-16.2038536990054));
#60273=CARTESIAN_POINT('Ctrl Pts',(-21.1624916905598,-18.1378073276301,
-16.2079669293832));
#60274=CARTESIAN_POINT('Ctrl Pts',(-21.1348035753301,-18.0594570997617,
-16.2120801597611));
#60275=CARTESIAN_POINT('Ctrl Pts',(-21.1033710027997,-17.9826285278121,
-16.2161933901389));
#60276=CARTESIAN_POINT('Ctrl Pts',(-21.0719418753926,-17.9058083765509,
-16.2203061696918));
#60277=CARTESIAN_POINT('Ctrl Pts',(-21.0367692860286,-17.830509988201,-16.2244189492448));
#60278=CARTESIAN_POINT('Ctrl Pts',(-20.998036835518,-17.757120421374,-16.2285317287978));
#60279=CARTESIAN_POINT('Ctrl Pts',(-20.9588192445656,-17.68281161896,-16.2326960226666));
#60280=CARTESIAN_POINT('Ctrl Pts',(-20.9159522062818,-17.610460238745,-16.2368603165354));
#60281=CARTESIAN_POINT('Ctrl Pts',(-20.8696736494984,-17.5404412648287,
-16.2410246104042));
#60282=CARTESIAN_POINT('Ctrl Pts',(-20.8239074514183,-17.4711974842889,
-16.2451428005836));
#60283=CARTESIAN_POINT('Ctrl Pts',(-20.7748052350545,-17.4042350697679,
-16.2492609907631));
#60284=CARTESIAN_POINT('Ctrl Pts',(-20.7226388747277,-17.3398847975651,
-16.2533791809425));
#60285=CARTESIAN_POINT('Ctrl Pts',(-20.6695965003384,-17.2744539105173,
-16.257566526656));
#60286=CARTESIAN_POINT('Ctrl Pts',(-20.6133864683218,-17.2117240820488,
-16.2617538723695));
#60287=CARTESIAN_POINT('Ctrl Pts',(-20.5543334369044,-17.152003839313,-16.265941218083));
#60288=CARTESIAN_POINT('Ctrl Pts',(-20.495280405487,-17.0922835965773,-16.2701285637965));
#60289=CARTESIAN_POINT('Ctrl Pts',(-20.4333847973435,-17.0355732283015,
-16.27431590951));
#60290=CARTESIAN_POINT('Ctrl Pts',(-20.369004471075,-16.9821369642625,-16.2785032552236));
#60291=CARTESIAN_POINT('Ctrl Pts',(-20.3046658312848,-16.9287353003847,
-16.2826878896166));
#60292=CARTESIAN_POINT('Ctrl Pts',(-20.2375884427954,-16.8783896656033,
-16.2868725240096));
#60293=CARTESIAN_POINT('Ctrl Pts',(-20.1680947292198,-16.8313934104545,
-16.2910571584027));
#60294=CARTESIAN_POINT('Ctrl Pts',(-20.0986999313439,-16.7844640486578,
-16.2952358364866));
#60295=CARTESIAN_POINT('Ctrl Pts',(-20.0268960178071,-16.740874852386,-16.2994145145706));
#60296=CARTESIAN_POINT('Ctrl Pts',(-19.9530388079927,-16.7008793047445,
-16.3035931926545));
#60297=CARTESIAN_POINT('Ctrl Pts',(-19.8778577607726,-16.6601668656558,
-16.30784677054));
#60298=CARTESIAN_POINT('Ctrl Pts',(-19.8005494535676,-16.623178482619,-16.3121003484254));
#60299=CARTESIAN_POINT('Ctrl Pts',(-19.7215205448425,-16.5901356572584,
-16.3163539263108));
#60300=CARTESIAN_POINT('Ctrl Pts',(-19.6440237657252,-16.5577334315453,
-16.3205250402888));
#60301=CARTESIAN_POINT('Ctrl Pts',(-19.5648729481498,-16.5291253296777,
-16.3246961542667));
#60302=CARTESIAN_POINT('Ctrl Pts',(-19.4844751811847,-16.5044732887207,
-16.3288672682447));
#60303=CARTESIAN_POINT('Ctrl Pts',(-19.4041043924668,-16.479829519994,-16.3330369825651));
#60304=CARTESIAN_POINT('Ctrl Pts',(-19.3224879248152,-16.4591393105013,
-16.3372066968854));
#60305=CARTESIAN_POINT('Ctrl Pts',(-19.2400494979669,-16.4425152111225,
-16.3413764112058));
#60306=CARTESIAN_POINT('Ctrl Pts',(-19.1576140046316,-16.4258917033006,
-16.3455459771499));
#60307=CARTESIAN_POINT('Ctrl Pts',(-19.0743570613776,-16.4133341080144,
-16.3497155430939));
#60308=CARTESIAN_POINT('Ctrl Pts',(-18.9907127437438,-16.404903895178,-16.3538851090379));
#60309=CARTESIAN_POINT('Ctrl Pts',(-18.9041275950884,-16.3961772864581,
-16.3582012717769));
#60310=CARTESIAN_POINT('Ctrl Pts',(-18.8171278498232,-16.3918737507556,
-16.3625174345158));
#60311=CARTESIAN_POINT('Ctrl Pts',(-18.7301989430816,-16.3920028218831,
-16.3668335972547));
#60312=CARTESIAN_POINT('Ctrl Pts',(-18.6461017363339,-16.3921276885323,
-16.3710091614464));
#60313=CARTESIAN_POINT('Ctrl Pts',(-18.5620712918896,-16.3964007414036,
-16.3751847256381));
#60314=CARTESIAN_POINT('Ctrl Pts',(-18.4785435740568,-16.4047775883437,
-16.3793602898298));
#60315=CARTESIAN_POINT('Ctrl Pts',(-18.3907970697645,-16.4135775299086,
-16.3837467518423));
#60316=CARTESIAN_POINT('Ctrl Pts',(-18.303605989369,-16.42690663756,-16.3881332138548));
#60317=CARTESIAN_POINT('Ctrl Pts',(-18.2174632822104,-16.4446528323395,
-16.3925196758674));
#60318=CARTESIAN_POINT('Ctrl Pts',(-18.1313205750518,-16.462399027119,-16.3969061378799));
#60319=CARTESIAN_POINT('Ctrl Pts',(-18.046226783443,-16.4845620891763,-16.4012925998925));
#60320=CARTESIAN_POINT('Ctrl Pts',(-17.9626538344087,-16.510970485056,-16.405679061905));
#60321=CARTESIAN_POINT('Ctrl Pts',(-17.8829440437002,-16.5361581532291,
-16.4098627597763));
#60322=CARTESIAN_POINT('Ctrl Pts',(-17.8043209701197,-16.5653010733625,
-16.4140464576476));
#60323=CARTESIAN_POINT('Ctrl Pts',(-17.7272055153423,-16.5982870043986,
-16.4182301555188));
#60324=CARTESIAN_POINT('Ctrl Pts',(-17.6501861873222,-16.6312318174695,
-16.4224086382836));
#60325=CARTESIAN_POINT('Ctrl Pts',(-17.5746711677127,-16.6680099558202,
-16.4265871210483));
#60326=CARTESIAN_POINT('Ctrl Pts',(-17.5010661413011,-16.708459472157,-16.4307656038131));
#60327=CARTESIAN_POINT('Ctrl Pts',(-17.4275438125226,-16.7488635421511,
-16.434939391917));
#60328=CARTESIAN_POINT('Ctrl Pts',(-17.3559276133303,-16.79293057247,-16.439113180021));
#60329=CARTESIAN_POINT('Ctrl Pts',(-17.2866017020174,-16.8404512397302,
-16.4432869681249));
#60330=CARTESIAN_POINT('Ctrl Pts',(-17.2485113698382,-16.8665609289797,
-16.4455802084489));
#60331=CARTESIAN_POINT('Ctrl Pts',(-17.2111120439232,-16.8937123832665,
-16.447873448773));
#60332=CARTESIAN_POINT('Ctrl Pts',(-17.1744641548914,-16.9218650419685,
-16.4501666890971));
#60333=CARTESIAN_POINT('Ctrl Pts',(-17.1721129765924,-16.9188350422745,
-15.6501589808892));
#60334=CARTESIAN_POINT('Ctrl Pts',(-16.5413044634767,-17.4084201550706,
-15.6900393300921));
#60335=CARTESIAN_POINT('Ctrl Pts',(-15.7364335242104,-19.0750467767261,
-15.7723116148555));
#60336=CARTESIAN_POINT('Ctrl Pts',(-17.1577428497044,-21.5363189092118,
-15.8969758351793));
#60337=CARTESIAN_POINT('Ctrl Pts',(-20.0538051259393,-21.6762256253679,
-16.0241516418607));
#60338=CARTESIAN_POINT('Ctrl Pts',(-21.2452320241039,-20.0081650284355,
-16.1140629935438));
#60339=CARTESIAN_POINT('Ctrl Pts',(-21.2975539525536,-19.0564768252052,
-16.1615824096664));
#60340=CARTESIAN_POINT('Ctrl Pts',(-21.2967673506771,-18.9536997966296,
-16.1667098902285));
#60341=CARTESIAN_POINT('Origin',(-18.734,-18.952,1.76670989022851));
#60342=CARTESIAN_POINT('',(-17.1744641548915,-16.9218650419685,-14.8500370269081));
#60343=CARTESIAN_POINT('',(-17.1744641548914,-16.9218650419685,-14.9167585796912));
#60344=CARTESIAN_POINT('',(-17.1744641548914,-16.9218650419685,1.76670989022851));
#60345=CARTESIAN_POINT('',(-21.293999428374,-18.9537107672548,-15.4332901097416));
#60346=CARTESIAN_POINT('Ctrl Pts',(-17.1744641548914,-16.9218650419685,
-14.9167585796912));
#60347=CARTESIAN_POINT('Ctrl Pts',(-17.1078480248072,-16.9730390992979,
-14.9209295740523));
#60348=CARTESIAN_POINT('Ctrl Pts',(-17.0437052951214,-17.0275323959551,
-14.9251005684134));
#60349=CARTESIAN_POINT('Ctrl Pts',(-16.9823783827407,-17.0850715841388,
-14.9292715627744));
#60350=CARTESIAN_POINT('Ctrl Pts',(-16.9210709423153,-17.1425925030105,
-14.9334412327999));
#60351=CARTESIAN_POINT('Ctrl Pts',(-16.8625778787664,-17.2031570781273,
-14.9376109028253));
#60352=CARTESIAN_POINT('Ctrl Pts',(-16.8072069412376,-17.2664530535447,
-14.9417805728507));
#60353=CARTESIAN_POINT('Ctrl Pts',(-16.7518369746777,-17.3297479190219,
-14.945950169758));
#60354=CARTESIAN_POINT('Ctrl Pts',(-16.6995893273772,-17.3957737426153,
-14.9501197666653));
#60355=CARTESIAN_POINT('Ctrl Pts',(-16.6507325015835,-17.4641839730526,
-14.9542893635725));
#60356=CARTESIAN_POINT('Ctrl Pts',(-16.6008932637074,-17.5339697950445,
-14.9585428026516));
#60357=CARTESIAN_POINT('Ctrl Pts',(-16.5545830040309,-17.6062365666551,
-14.9627962417306));
#60358=CARTESIAN_POINT('Ctrl Pts',(-16.512040211465,-17.6805855521767,-14.9670496808097));
#60359=CARTESIAN_POINT('Ctrl Pts',(-16.4702752098586,-17.7535752482561,
-14.9712253561534));
#60360=CARTESIAN_POINT('Ctrl Pts',(-16.4321412272479,-17.8285712145274,
-14.9754010314971));
#60361=CARTESIAN_POINT('Ctrl Pts',(-16.397816458658,-17.905173146522,-14.9795767068408));
#60362=CARTESIAN_POINT('Ctrl Pts',(-16.3625328431747,-17.9839149188573,
-14.9838690277875));
#60363=CARTESIAN_POINT('Ctrl Pts',(-16.3312746199873,-18.0643532285809,
-14.9881613487342));
#60364=CARTESIAN_POINT('Ctrl Pts',(-16.3041808697538,-18.1460353641197,
-14.9924536696809));
#60365=CARTESIAN_POINT('Ctrl Pts',(-16.2770871195203,-18.2277174996585,
-14.9967459906277));
#60366=CARTESIAN_POINT('Ctrl Pts',(-16.2541579140775,-18.3106429409755,
-15.0010383115744));
#60367=CARTESIAN_POINT('Ctrl Pts',(-16.2354754819719,-18.3943484665023,
-15.0053306325211));
#60368=CARTESIAN_POINT('Ctrl Pts',(-16.21726175823,-18.4759539720913,-15.0095152669141));
#60369=CARTESIAN_POINT('Ctrl Pts',(-16.2030163785017,-18.5586046111965,
-15.0136999013072));
#60370=CARTESIAN_POINT('Ctrl Pts',(-16.1928535263697,-18.6418797014761,
-15.0178845357002));
#60371=CARTESIAN_POINT('Ctrl Pts',(-16.1827051397999,-18.7250362599721,
-15.0220632137842));
#60372=CARTESIAN_POINT('Ctrl Pts',(-16.1766277936582,-18.8088150514093,
-15.0262418918681));
#60373=CARTESIAN_POINT('Ctrl Pts',(-16.1746849654928,-18.8927838354389,
-15.0304205699521));
#60374=CARTESIAN_POINT('Ctrl Pts',(-16.1727073135288,-18.978257699575,-15.0346741478375));
#60375=CARTESIAN_POINT('Ctrl Pts',(-16.1750139649456,-19.0639279639718,
-15.0389277257229));
#60376=CARTESIAN_POINT('Ctrl Pts',(-16.1816167614736,-19.149331709792,-15.0431813036084));
#60377=CARTESIAN_POINT('Ctrl Pts',(-16.1880915499065,-19.2330797373478,
-15.0473524175863));
#60378=CARTESIAN_POINT('Ctrl Pts',(-16.1986973545604,-19.3165710082866,
-15.0515235315643));
#60379=CARTESIAN_POINT('Ctrl Pts',(-16.2133928011124,-19.3993693651964,
-15.0556946455422));
#60380=CARTESIAN_POINT('Ctrl Pts',(-16.2280833164655,-19.4821399383179,
-15.0598643598626));
#60381=CARTESIAN_POINT('Ctrl Pts',(-16.2468606679443,-19.5642176066097,
-15.064034074183));
#60382=CARTESIAN_POINT('Ctrl Pts',(-16.2696319425036,-19.6451739155444,
-15.0682037885034));
#60383=CARTESIAN_POINT('Ctrl Pts',(-16.2924024067631,-19.7261273437063,
-15.0723733544474));
#60384=CARTESIAN_POINT('Ctrl Pts',(-16.3191663861463,-19.8059590492309,
-15.0765429203915));
#60385=CARTESIAN_POINT('Ctrl Pts',(-16.3497807798976,-19.8842546382263,
-15.0807124863355));
#60386=CARTESIAN_POINT('Ctrl Pts',(-16.3814715379663,-19.9653030035427,
-15.0850286490744));
#60387=CARTESIAN_POINT('Ctrl Pts',(-16.4172883172413,-20.0447047315976,
-15.0893448118133));
#60388=CARTESIAN_POINT('Ctrl Pts',(-16.4570183818636,-20.1220233803942,
-15.0936609745523));
#60389=CARTESIAN_POINT('Ctrl Pts',(-16.4954542438098,-20.1968233823387,
-15.0978365387439));
#60390=CARTESIAN_POINT('Ctrl Pts',(-16.5375520792277,-20.2696735493081,
-15.1020121029356));
#60391=CARTESIAN_POINT('Ctrl Pts',(-16.583073696292,-20.3402060495535,-15.1061876671273));
#60392=CARTESIAN_POINT('Ctrl Pts',(-16.6308945020167,-20.4143009787112,
-15.1105741291398));
#60393=CARTESIAN_POINT('Ctrl Pts',(-16.6824937078808,-20.4858374838362,
-15.1149605911524));
#60394=CARTESIAN_POINT('Ctrl Pts',(-16.7375469032625,-20.5544278556388,
-15.1193470531649));
#60395=CARTESIAN_POINT('Ctrl Pts',(-16.7926000986442,-20.6230182274414,
-15.1237335151774));
#60396=CARTESIAN_POINT('Ctrl Pts',(-16.851106840707,-20.6886620833861,-15.12811997719));
#60397=CARTESIAN_POINT('Ctrl Pts',(-16.9126993772538,-20.7510175211999,
-15.1325064392025));
#60398=CARTESIAN_POINT('Ctrl Pts',(-16.9714579498921,-20.810503892887,-15.1366910735956));
#60399=CARTESIAN_POINT('Ctrl Pts',(-17.0332433037704,-20.8672192262126,
-15.1408757079886));
#60400=CARTESIAN_POINT('Ctrl Pts',(-17.0977635170215,-20.9208398034807,
-15.1450603423817));
#60401=CARTESIAN_POINT('Ctrl Pts',(-17.162191893735,-20.9743840584939,-15.1492390204656));
#60402=CARTESIAN_POINT('Ctrl Pts',(-17.2293470468519,-21.0248420156528,
-15.1534176985496));
#60403=CARTESIAN_POINT('Ctrl Pts',(-17.2988998898354,-21.0719263368819,
-15.1575963766335));
#60404=CARTESIAN_POINT('Ctrl Pts',(-17.3696994175427,-21.1198546107302,
-15.1618499545189));
#60405=CARTESIAN_POINT('Ctrl Pts',(-17.4429830989499,-21.1642867711771,
-15.1661035324044));
#60406=CARTESIAN_POINT('Ctrl Pts',(-17.5183681022775,-21.2049622920146,
-15.1703571102898));
#60407=CARTESIAN_POINT('Ctrl Pts',(-17.5922916202138,-21.2448492385089,
-15.1745282242678));
#60408=CARTESIAN_POINT('Ctrl Pts',(-17.6682352871973,-21.281123676622,-15.1786993382457));
#60409=CARTESIAN_POINT('Ctrl Pts',(-17.7458099687318,-21.3135843118767,
-15.1828704522237));
#60410=CARTESIAN_POINT('Ctrl Pts',(-17.8233586193327,-21.3460340546518,
-15.187040166544));
#60411=CARTESIAN_POINT('Ctrl Pts',(-17.9025367735084,-21.3746723587587,
-15.1912098808644));
#60412=CARTESIAN_POINT('Ctrl Pts',(-17.9829338767364,-21.3993454350553,
-15.1953795951848));
#60413=CARTESIAN_POINT('Ctrl Pts',(-18.0633281190904,-21.4240176333778,
-15.1995491611289));
#60414=CARTESIAN_POINT('Ctrl Pts',(-18.1449407842163,-21.4447247502805,
-15.2037187270729));
#60415=CARTESIAN_POINT('Ctrl Pts',(-18.2273459747055,-21.4613628072985,
-15.2078882930169));
#60416=CARTESIAN_POINT('Ctrl Pts',(-18.3126484300345,-21.4785858378759,
-15.2122044557559));
#60417=CARTESIAN_POINT('Ctrl Pts',(-18.3987996610354,-21.4914482440571,
-15.2165206184948));
#60418=CARTESIAN_POINT('Ctrl Pts',(-18.4853175391717,-21.4998926652582,
-15.2208367812337));
#60419=CARTESIAN_POINT('Ctrl Pts',(-18.5690171065278,-21.5080620103268,
-15.2250123454254));
#60420=CARTESIAN_POINT('Ctrl Pts',(-18.6530593280231,-21.512096806535,-15.2291879096171));
#60421=CARTESIAN_POINT('Ctrl Pts',(-18.7370059866504,-21.5119982351643,
-15.2333634738087));
#60422=CARTESIAN_POINT('Ctrl Pts',(-18.8251925914409,-21.5118946851879,
-15.2377499358213));
#60423=CARTESIAN_POINT('Ctrl Pts',(-18.9132731428316,-21.5072292722347,
-15.2421363978338));
#60424=CARTESIAN_POINT('Ctrl Pts',(-19.0007460413497,-21.4980649146132,
-15.2465228598464));
#60425=CARTESIAN_POINT('Ctrl Pts',(-19.0882189398678,-21.4889005569917,
-15.2509093218589));
#60426=CARTESIAN_POINT('Ctrl Pts',(-19.1750836241625,-21.4752374199982,
-15.2552957838715));
#60427=CARTESIAN_POINT('Ctrl Pts',(-19.2608535512399,-21.4571996598167,
-15.259682245884));
#60428=CARTESIAN_POINT('Ctrl Pts',(-19.3426770768309,-21.4399918437197,
-15.263866880277));
#60429=CARTESIAN_POINT('Ctrl Pts',(-19.4238089369639,-21.4187390730901,
-15.2680515146701));
#60430=CARTESIAN_POINT('Ctrl Pts',(-19.5038189245161,-21.3935115857716,
-15.2722361490631));
#60431=CARTESIAN_POINT('Ctrl Pts',(-19.5837150277544,-21.3683200066587,
-15.2764148271471));
#60432=CARTESIAN_POINT('Ctrl Pts',(-19.6624919952641,-21.33916508562,-15.280593505231));
#60433=CARTESIAN_POINT('Ctrl Pts',(-19.7397300928954,-21.3061680017035,
-15.284772183315));
#60434=CARTESIAN_POINT('Ctrl Pts',(-19.8183526279167,-21.2725794687723,
-15.2890257612004));
#60435=CARTESIAN_POINT('Ctrl Pts',(-19.8953801101215,-21.2350097758302,
-15.2932793390858));
#60436=CARTESIAN_POINT('Ctrl Pts',(-19.9703862586167,-21.1936398059242,
-15.2975329169713));
#60437=CARTESIAN_POINT('Ctrl Pts',(-20.0439382665608,-21.1530718736117,
-15.3017040309492));
#60438=CARTESIAN_POINT('Ctrl Pts',(-20.1155461950122,-21.1088499333759,
-15.3058751449272));
#60439=CARTESIAN_POINT('Ctrl Pts',(-20.1848301560489,-21.0611922288637,
-15.3100462589051));
#60440=CARTESIAN_POINT('Ctrl Pts',(-20.2540908681833,-21.0135505163546,
-15.3142159732255));
#60441=CARTESIAN_POINT('Ctrl Pts',(-20.3210287829501,-20.9624755897522,
-15.3183856875459));
#60442=CARTESIAN_POINT('Ctrl Pts',(-20.385292362642,-20.9082294172924,-15.3225554018662));
#60443=CARTESIAN_POINT('Ctrl Pts',(-20.4495536555601,-20.8539851751441,
-15.3267249678103));
#60444=CARTESIAN_POINT('Ctrl Pts',(-20.5111404516291,-20.7965702088954,
-15.3308945337543));
#60445=CARTESIAN_POINT('Ctrl Pts',(-20.5697347912254,-20.7362863492962,
-15.3350640996984));
#60446=CARTESIAN_POINT('Ctrl Pts',(-20.630389235518,-20.6738829835616,-15.3393802624373));
#60447=CARTESIAN_POINT('Ctrl Pts',(-20.68783651095,-20.6084056085287,-15.3436964251762));
#60448=CARTESIAN_POINT('Ctrl Pts',(-20.7417674193154,-20.540228569802,-15.3480125879152));
#60449=CARTESIAN_POINT('Ctrl Pts',(-20.7939415340134,-20.474272390941,-15.3521881521068));
#60450=CARTESIAN_POINT('Ctrl Pts',(-20.8428246196129,-20.4057901412947,
-15.3563637162985));
#60451=CARTESIAN_POINT('Ctrl Pts',(-20.8881804708301,-20.3351509314223,
-15.3605392804902));
#60452=CARTESIAN_POINT('Ctrl Pts',(-20.9358271382689,-20.2609439029881,
-15.3649257425027));
#60453=CARTESIAN_POINT('Ctrl Pts',(-20.9795805961809,-20.1843567987729,
-15.3693122045153));
#60454=CARTESIAN_POINT('Ctrl Pts',(-21.0192222426254,-20.1058454410407,
-15.3736986665278));
#60455=CARTESIAN_POINT('Ctrl Pts',(-21.0588638890698,-20.0273340833085,
-15.3780851285404));
#60456=CARTESIAN_POINT('Ctrl Pts',(-21.0943935591863,-19.9468990335382,
-15.3824715905529));
#60457=CARTESIAN_POINT('Ctrl Pts',(-21.1256522921828,-19.8650166007783,
-15.3868580525655));
#60458=CARTESIAN_POINT('Ctrl Pts',(-21.1596866697226,-19.7758633510054,
-15.3916340140293));
#60459=CARTESIAN_POINT('Ctrl Pts',(-21.1887650239783,-19.6847190703918,
-15.3964099754931));
#60460=CARTESIAN_POINT('Ctrl Pts',(-21.2126811308614,-19.5921092496689,
-15.4011859369569));
#60461=CARTESIAN_POINT('Ctrl Pts',(-21.2364993763692,-19.4998783754223,
-15.4059423558521));
#60462=CARTESIAN_POINT('Ctrl Pts',(-21.2551974088384,-19.4061941121839,
-15.4106987747474));
#60463=CARTESIAN_POINT('Ctrl Pts',(-21.2686182636666,-19.3115973546727,
-15.4154551936427));
#60464=CARTESIAN_POINT('Ctrl Pts',(-21.2819450244391,-19.2176638181475,
-15.4201782651282));
#60465=CARTESIAN_POINT('Ctrl Pts',(-21.2900682365862,-19.1228307363249,
-15.4249013366138));
#60466=CARTESIAN_POINT('Ctrl Pts',(-21.2928821031965,-19.0276464271503,
-15.4296244080994));
#60467=CARTESIAN_POINT('Ctrl Pts',(-21.2936100754836,-19.0030214008636,
-15.4308463086468));
#60468=CARTESIAN_POINT('Ctrl Pts',(-21.2939829474075,-18.9783729560409,
-15.4320682091942));
#60469=CARTESIAN_POINT('Ctrl Pts',(-21.293999428374,-18.9537107672549,-15.4332901097416));
#60470=CARTESIAN_POINT('Ctrl Pts',(-21.2939994283744,-18.9537107666516,
-15.4332901097715));
#60471=CARTESIAN_POINT('Ctrl Pts',(-21.2940559692553,-18.8691027211111,
-15.437482057942));
#60472=CARTESIAN_POINT('Ctrl Pts',(-21.2899137324165,-18.7844696898645,
-15.4416740061124));
#60473=CARTESIAN_POINT('Ctrl Pts',(-21.2815918669692,-18.7002547332074,
-15.4458659542829));
#60474=CARTESIAN_POINT('Ctrl Pts',(-21.2732695913204,-18.6160356254257,
-15.4500581090829));
#60475=CARTESIAN_POINT('Ctrl Pts',(-21.2607673227297,-18.5322350838833,
-15.4542502638829));
#60476=CARTESIAN_POINT('Ctrl Pts',(-21.2441560631151,-18.449290800953,-15.4584424186829));
#60477=CARTESIAN_POINT('Ctrl Pts',(-21.2275392030056,-18.3663185533138,
-15.4626359868701));
#60478=CARTESIAN_POINT('Ctrl Pts',(-21.2068106889621,-18.2842035816671,
-15.4668295550574));
#60479=CARTESIAN_POINT('Ctrl Pts',(-21.1820923104735,-18.2033718951306,
-15.4710231232446));
#60480=CARTESIAN_POINT('Ctrl Pts',(-21.1573415752886,-18.1224343988081,
-15.4752221808701));
#60481=CARTESIAN_POINT('Ctrl Pts',(-21.1285906849035,-18.0427839738201,
-15.4794212384956));
#60482=CARTESIAN_POINT('Ctrl Pts',(-21.0960107310926,-17.9648296468171,
-15.483620296121));
#60483=CARTESIAN_POINT('Ctrl Pts',(-21.0634063961442,-17.8868169828631,
-15.4878224961022));
#60484=CARTESIAN_POINT('Ctrl Pts',(-21.0269674888688,-17.8105033515339,
-15.4920246960833));
#60485=CARTESIAN_POINT('Ctrl Pts',(-20.9869114421218,-17.7362738655615,
-15.4962268960644));
#60486=CARTESIAN_POINT('Ctrl Pts',(-20.9467843119657,-17.6619126520388,
-15.5004365532642));
#60487=CARTESIAN_POINT('Ctrl Pts',(-20.9030274638811,-17.5896433529156,
-15.5046462104641));
#60488=CARTESIAN_POINT('Ctrl Pts',(-20.8559018807132,-17.5198224940232,
-15.5088558676639));
#60489=CARTESIAN_POINT('Ctrl Pts',(-20.8365799691019,-17.4911953158865,
-15.5105818648582));
#60490=CARTESIAN_POINT('Ctrl Pts',(-20.8166922183615,-17.4629793510679,
-15.5123078620525));
#60491=CARTESIAN_POINT('Ctrl Pts',(-20.7962584977301,-17.435197478727,-15.5140338592469));
#60492=CARTESIAN_POINT('Ctrl Pts',(-20.7467174843303,-17.3678410665132,
-15.5182184936399));
#60493=CARTESIAN_POINT('Ctrl Pts',(-20.6937808669812,-17.3027889832896,
-15.522403128033));
#60494=CARTESIAN_POINT('Ctrl Pts',(-20.6376906991394,-17.2404037502932,
-15.526587762426));
#60495=CARTESIAN_POINT('Ctrl Pts',(-20.581680368709,-17.1781073149544,-15.53076644051));
#60496=CARTESIAN_POINT('Ctrl Pts',(-20.522525708678,-17.1184705290968,-15.5349451185939));
#60497=CARTESIAN_POINT('Ctrl Pts',(-20.4605108062944,-17.061825289623,-15.5391237966778));
#60498=CARTESIAN_POINT('Ctrl Pts',(-20.3973843313549,-17.0041647249419,
-15.5433773745633));
#60499=CARTESIAN_POINT('Ctrl Pts',(-20.3312943514667,-16.9496043968549,
-15.5476309524487));
#60500=CARTESIAN_POINT('Ctrl Pts',(-20.2625820107878,-16.8984574422973,
-15.5518845303342));
#60501=CARTESIAN_POINT('Ctrl Pts',(-20.195201792914,-16.8483020712589,-15.5560556443121));
#60502=CARTESIAN_POINT('Ctrl Pts',(-20.1253003720614,-16.8014291923403,
-15.5602267582901));
#60503=CARTESIAN_POINT('Ctrl Pts',(-20.0532336923064,-16.7580942442567,
-15.564397872268));
#60504=CARTESIAN_POINT('Ctrl Pts',(-19.9811911952218,-16.7147738376335,
-15.5685675865884));
#60505=CARTESIAN_POINT('Ctrl Pts',(-19.9069852761389,-16.6749892409427,
-15.5727373009088));
#60506=CARTESIAN_POINT('Ctrl Pts',(-19.8309999421957,-16.6389519834594,
-15.5769070152291));
#60507=CARTESIAN_POINT('Ctrl Pts',(-19.7550173121369,-16.6029160083363,
-15.5810765811732));
#60508=CARTESIAN_POINT('Ctrl Pts',(-19.6772558091333,-16.5706273036551,
-15.5852461471172));
#60509=CARTESIAN_POINT('Ctrl Pts',(-19.5981218233864,-16.5422503295265,
-15.5894157130613));
#60510=CARTESIAN_POINT('Ctrl Pts',(-19.516205584323,-16.5128756559943,-15.5937318758002));
#60511=CARTESIAN_POINT('Ctrl Pts',(-19.4328190502828,-16.4876930819298,
-15.5980480385391));
#60512=CARTESIAN_POINT('Ctrl Pts',(-19.3484309915969,-16.4668290689441,
-15.602364201278));
#60513=CARTESIAN_POINT('Ctrl Pts',(-19.2667918650467,-16.4466446989869,
-15.6065397654697));
#60514=CARTESIAN_POINT('Ctrl Pts',(-19.1842159325102,-16.4305019005906,
-15.6107153296614));
#60515=CARTESIAN_POINT('Ctrl Pts',(-19.1011369778116,-16.4184628600466,
-15.6148908938531));
#60516=CARTESIAN_POINT('Ctrl Pts',(-19.0138619026128,-16.4058157561848,
-15.6192773558656));
#60517=CARTESIAN_POINT('Ctrl Pts',(-18.926032235907,-16.3976979204099,-15.6236638178781));
#60518=CARTESIAN_POINT('Ctrl Pts',(-18.8381534037014,-16.3941196141146,
-15.6280502798907));
#60519=CARTESIAN_POINT('Ctrl Pts',(-18.7502745714958,-16.3905413078192,
-15.6324367419032));
#60520=CARTESIAN_POINT('Ctrl Pts',(-18.6623471531412,-16.391502448601,-15.6368232039158));
#60521=CARTESIAN_POINT('Ctrl Pts',(-18.5748705298081,-16.3969505265619,
-15.6412096659283));
#60522=CARTESIAN_POINT('Ctrl Pts',(-18.4914284406973,-16.4021473321697,
-15.6453938186789));
#60523=CARTESIAN_POINT('Ctrl Pts',(-18.4080859286891,-16.4114456475977,
-15.6495779714295));
#60524=CARTESIAN_POINT('Ctrl Pts',(-18.3252786851494,-16.4248381755838,
-15.6537621241801));
#60525=CARTESIAN_POINT('Ctrl Pts',(-18.2425831161189,-16.4382126422997,
-15.6579406341489));
#60526=CARTESIAN_POINT('Ctrl Pts',(-18.1604218322578,-16.4556702853485,
-15.6621191441177));
#60527=CARTESIAN_POINT('Ctrl Pts',(-18.0792276257711,-16.477151895985,-15.6662976540865));
#60528=CARTESIAN_POINT('Ctrl Pts',(-17.997681334868,-16.4987266578532,-15.67049428343));
#60529=CARTESIAN_POINT('Ctrl Pts',(-17.9171109977116,-16.5243603430073,
-15.6746909127734));
#60530=CARTESIAN_POINT('Ctrl Pts',(-17.8379469013808,-16.5539406086473,
-15.6788875421169));
#60531=CARTESIAN_POINT('Ctrl Pts',(-17.7592670966102,-16.5833399150688,
-15.6830584983046));
#60532=CARTESIAN_POINT('Ctrl Pts',(-17.6819768120108,-16.6166374905021,
-15.6872294544923));
#60533=CARTESIAN_POINT('Ctrl Pts',(-17.6064837009691,-16.6536730007634,
-15.69140041068));
#60534=CARTESIAN_POINT('Ctrl Pts',(-17.5302935747919,-16.6910504536318,
-15.6956098766013));
#60535=CARTESIAN_POINT('Ctrl Pts',(-17.4559344312179,-16.7322350696159,
-15.6998193425226));
#60536=CARTESIAN_POINT('Ctrl Pts',(-17.383803351038,-16.777012871502,-15.7040288084439));
#60537=CARTESIAN_POINT('Ctrl Pts',(-17.3116722708582,-16.8217906733882,
-15.7082382743652));
#60538=CARTESIAN_POINT('Ctrl Pts',(-17.2417696646533,-16.8701614078669,
-15.7124477402865));
#60539=CARTESIAN_POINT('Ctrl Pts',(-17.1744641548914,-16.9218650419685,
-15.7166572062078));
#60540=CARTESIAN_POINT('',(-21.2939991231355,-18.9498811452879,-15.3667098902285));
#60541=CARTESIAN_POINT('Ctrl Pts',(-21.2956373739999,-18.9498797893439,
-15.3667098902285));
#60542=CARTESIAN_POINT('Ctrl Pts',(-21.296922788715,-18.8056440679786,-15.3738974629702));
#60543=CARTESIAN_POINT('Ctrl Pts',(-21.2201491749354,-17.8120820090192,
-15.4234769712724));
#60544=CARTESIAN_POINT('Ctrl Pts',(-19.9200692397814,-16.166945137558,-15.515448415135));
#60545=CARTESIAN_POINT('Ctrl Pts',(-17.9391679634644,-16.3593206301496,
-15.6027438726135));
#60546=CARTESIAN_POINT('Ctrl Pts',(-17.2118400624246,-16.888001929858,-15.6476473945316));
#60547=CARTESIAN_POINT('Ctrl Pts',(-17.1721129765924,-16.9188350422745,
-15.6501589808892));
#60548=CARTESIAN_POINT('Ctrl Pts',(-17.1744641548915,-16.9218650419685,
-14.8500370269081));
#60549=CARTESIAN_POINT('Ctrl Pts',(-17.1078234648678,-16.9730579660761,
-14.8542147166677));
#60550=CARTESIAN_POINT('Ctrl Pts',(-17.0437722116886,-17.0274847849136,
-14.8583924064273));
#60551=CARTESIAN_POINT('Ctrl Pts',(-16.98262429975,-17.0848408861123,-14.8625700961868));
#60552=CARTESIAN_POINT('Ctrl Pts',(-16.9213774940062,-17.142289748665,-14.8667545424754));
#60553=CARTESIAN_POINT('Ctrl Pts',(-16.8630437183746,-17.2026770171266,
-14.8709389887639));
#60554=CARTESIAN_POINT('Ctrl Pts',(-16.8078981185104,-17.2656632773606,
-14.8751234350524));
#60555=CARTESIAN_POINT('Ctrl Pts',(-16.7883675060572,-17.2879707731814,
-14.8766054172776));
#60556=CARTESIAN_POINT('Ctrl Pts',(-16.7692364062925,-17.3106039888822,
-14.8780873995027));
#60557=CARTESIAN_POINT('Ctrl Pts',(-16.7505157350919,-17.3335469821889,
-14.8795693817278));
#60558=CARTESIAN_POINT('Ctrl Pts',(-16.6976546661539,-17.398330511467,-14.8837540161209));
#60559=CARTESIAN_POINT('Ctrl Pts',(-16.6478724513803,-17.4658271045687,
-14.8879386505139));
#60560=CARTESIAN_POINT('Ctrl Pts',(-16.6014597312929,-17.5357118928894,
-14.892123284907));
#60561=CARTESIAN_POINT('Ctrl Pts',(-16.5551130739679,-17.605497208864,-14.8963019629909));
#60562=CARTESIAN_POINT('Ctrl Pts',(-16.5121266371781,-17.6776635880369,
-14.9004806410749));
#60563=CARTESIAN_POINT('Ctrl Pts',(-16.4727509157818,-17.7518531010238,
-14.9046593191588));
#60564=CARTESIAN_POINT('Ctrl Pts',(-16.4326694128783,-17.8273724077119,
-14.9089128970443));
#60565=CARTESIAN_POINT('Ctrl Pts',(-16.3963296475342,-17.9049877173956,
-14.9131664749297));
#60566=CARTESIAN_POINT('Ctrl Pts',(-16.3639497085597,-17.98429053118,-14.9174200528151));
#60567=CARTESIAN_POINT('Ctrl Pts',(-16.3321975178866,-18.0620559051724,
-14.9215911667931));
#60568=CARTESIAN_POINT('Ctrl Pts',(-16.3042531677127,-18.1414434905287,
-14.925762280771));
#60569=CARTESIAN_POINT('Ctrl Pts',(-16.2802751807717,-18.2220448565132,
-14.929933394749));
#60570=CARTESIAN_POINT('Ctrl Pts',(-16.2563052398757,-18.302619175931,-14.9341031090694));
#60571=CARTESIAN_POINT('Ctrl Pts',(-16.2362991499856,-18.3844060265128,
-14.9382728233897));
#60572=CARTESIAN_POINT('Ctrl Pts',(-16.2203659101291,-18.4669807609602,
-14.9424425377101));
#60573=CARTESIAN_POINT('Ctrl Pts',(-16.2044332372455,-18.5495525570442,
-14.9466121036542));
#60574=CARTESIAN_POINT('Ctrl Pts',(-16.1925732125598,-18.6329117293879,
-14.9507816695982));
#60575=CARTESIAN_POINT('Ctrl Pts',(-16.1848436692123,-18.7166237029672,
-14.9549512355423));
#60576=CARTESIAN_POINT('Ctrl Pts',(-16.1768423646561,-18.8032788862675,
-14.9592673982812));
#60577=CARTESIAN_POINT('Ctrl Pts',(-16.1732674495782,-18.890311616191,-14.9635835610201));
#60578=CARTESIAN_POINT('Ctrl Pts',(-16.1741243927921,-18.9772363947927,
-14.967899723759));
#60579=CARTESIAN_POINT('Ctrl Pts',(-16.174953421171,-19.0613296078744,-14.9720752879507));
#60580=CARTESIAN_POINT('Ctrl Pts',(-16.1799299313356,-19.1453213272336,
-14.9762508521424));
#60581=CARTESIAN_POINT('Ctrl Pts',(-16.1890058822549,-19.228775975552,-14.9804264163341));
#60582=CARTESIAN_POINT('Ctrl Pts',(-16.1985402378791,-19.3164457197621,
-14.9848128783466));
#60583=CARTESIAN_POINT('Ctrl Pts',(-16.2125989501167,-19.4035221357512,
-14.9891993403591));
#60584=CARTESIAN_POINT('Ctrl Pts',(-16.2310658163555,-19.4895132299243,
-14.9935858023717));
#60585=CARTESIAN_POINT('Ctrl Pts',(-16.2495326825942,-19.5755043240973,
-14.9979722643842));
#60586=CARTESIAN_POINT('Ctrl Pts',(-16.2724074784503,-19.660409556001,-15.0023587263968));
#60587=CARTESIAN_POINT('Ctrl Pts',(-16.2995147249235,-19.7437584514457,
-15.0067451884093));
#60588=CARTESIAN_POINT('Ctrl Pts',(-16.325374726804,-19.8232723406583,-15.0109298228023));
#60589=CARTESIAN_POINT('Ctrl Pts',(-16.3551825113724,-19.9016659307484,
-15.0151144571954));
#60590=CARTESIAN_POINT('Ctrl Pts',(-16.3888222337461,-19.9785189938177,
-15.0192990915884));
#60591=CARTESIAN_POINT('Ctrl Pts',(-16.4224140741388,-20.0552626660643,
-15.0234777696724));
#60592=CARTESIAN_POINT('Ctrl Pts',(-16.459826835514,-20.130469748956,-15.0276564477563));
#60593=CARTESIAN_POINT('Ctrl Pts',(-16.5008951440188,-20.2037358755717,
-15.0318351258403));
#60594=CARTESIAN_POINT('Ctrl Pts',(-16.5426995724383,-20.2783152448515,
-15.0360887037257));
#60595=CARTESIAN_POINT('Ctrl Pts',(-16.5882917392507,-20.3508829316544,
-15.0403422816111));
#60596=CARTESIAN_POINT('Ctrl Pts',(-16.6374462088682,-20.4210344451002,
-15.0445958594966));
#60597=CARTESIAN_POINT('Ctrl Pts',(-16.6856477231751,-20.4898259345683,
-15.0487669734745));
#60598=CARTESIAN_POINT('Ctrl Pts',(-16.7372743723593,-20.5562937050238,
-15.0529380874525));
#60599=CARTESIAN_POINT('Ctrl Pts',(-16.7920685361568,-20.6200833881242,
-15.0571092014304));
#60600=CARTESIAN_POINT('Ctrl Pts',(-16.8468443132435,-20.6838516659803,
-15.0612789157508));
#60601=CARTESIAN_POINT('Ctrl Pts',(-16.9047851945211,-20.744943292555,-15.0654486300712));
#60602=CARTESIAN_POINT('Ctrl Pts',(-16.9655931179196,-20.8030367633872,
-15.0696183443915));
#60603=CARTESIAN_POINT('Ctrl Pts',(-17.0263988775113,-20.8611281670043,
-15.0737879103356));
#60604=CARTESIAN_POINT('Ctrl Pts',(-17.090071143158,-20.9162213098333,-15.0779574762796));
#60605=CARTESIAN_POINT('Ctrl Pts',(-17.1562758100195,-20.9680323361371,
-15.0821270422237));
#60606=CARTESIAN_POINT('Ctrl Pts',(-17.2248081512956,-21.02166497421,-15.0864432049626));
#60607=CARTESIAN_POINT('Ctrl Pts',(-17.2960538702051,-21.0717800780493,
-15.0907593677015));
#60608=CARTESIAN_POINT('Ctrl Pts',(-17.3696076999733,-21.118110258419,-15.0950755304404));
#60609=CARTESIAN_POINT('Ctrl Pts',(-17.4407655214732,-21.1629312380361,
-15.0992510946321));
#60610=CARTESIAN_POINT('Ctrl Pts',(-17.5140829560416,-21.2042099051977,
-15.1034266588238));
#60611=CARTESIAN_POINT('Ctrl Pts',(-17.5891677483864,-21.241750885067,-15.1076022230155));
#60612=CARTESIAN_POINT('Ctrl Pts',(-17.6680448950955,-21.2811879705844,
-15.111988685028));
#60613=CARTESIAN_POINT('Ctrl Pts',(-17.7488720950907,-21.3164996308722,
-15.1163751470406));
#60614=CARTESIAN_POINT('Ctrl Pts',(-17.831172761348,-21.3475172671363,-15.1207616090531));
#60615=CARTESIAN_POINT('Ctrl Pts',(-17.9134734276052,-21.3785349034003,
-15.1251480710657));
#60616=CARTESIAN_POINT('Ctrl Pts',(-17.9972469842344,-21.4052584117747,
-15.1295345330782));
#60617=CARTESIAN_POINT('Ctrl Pts',(-18.0820028534413,-21.4275806835729,
-15.1339209950908));
#60618=CARTESIAN_POINT('Ctrl Pts',(-18.1628589794675,-21.4488758745561,
-15.1381056294838));
#60619=CARTESIAN_POINT('Ctrl Pts',(-18.2449099711163,-21.4662452083818,
-15.1422902638769));
#60620=CARTESIAN_POINT('Ctrl Pts',(-18.3277397785898,-21.4795586308728,
-15.1464748982699));
#60621=CARTESIAN_POINT('Ctrl Pts',(-18.4104516880846,-21.4928531033548,
-15.1506535763538));
#60622=CARTESIAN_POINT('Ctrl Pts',(-18.4939397611609,-21.5021030592902,
-15.1548322544378));
#60623=CARTESIAN_POINT('Ctrl Pts',(-18.5777744755002,-21.5072286757734,
-15.1590109325217));
#60624=CARTESIAN_POINT('Ctrl Pts',(-18.6631118668432,-21.5124461652484,
-15.1632645104072));
#60625=CARTESIAN_POINT('Ctrl Pts',(-18.7488079825307,-21.5133898805874,
-15.1675180882926));
#60626=CARTESIAN_POINT('Ctrl Pts',(-18.8344006857365,-21.510030434202,-15.171771666178));
#60627=CARTESIAN_POINT('Ctrl Pts',(-18.9183340073703,-21.5067361172402,
-15.175942780156));
#60628=CARTESIAN_POINT('Ctrl Pts',(-19.0021674095972,-21.4993040188572,
-15.1801138941339));
#60629=CARTESIAN_POINT('Ctrl Pts',(-19.0854634797585,-21.4877589440631,
-15.1842850081119));
#60630=CARTESIAN_POINT('Ctrl Pts',(-19.1687315991189,-21.4762177433303,
-15.1884547224322));
#60631=CARTESIAN_POINT('Ctrl Pts',(-19.2514622892086,-21.4605663702897,
-15.1926244367526));
#60632=CARTESIAN_POINT('Ctrl Pts',(-19.3332238803095,-21.4408814237056,
-15.196794151073));
#60633=CARTESIAN_POINT('Ctrl Pts',(-19.4149825619821,-21.4211971775964,
-15.200963717017));
#60634=CARTESIAN_POINT('Ctrl Pts',(-19.495771766177,-21.3974797518312,-15.2051332829611));
#60635=CARTESIAN_POINT('Ctrl Pts',(-19.5751719705271,-21.3698564299808,
-15.2093028489051));
#60636=CARTESIAN_POINT('Ctrl Pts',(-19.6573637881113,-21.3412619062112,
-15.213619011644));
#60637=CARTESIAN_POINT('Ctrl Pts',(-19.7380666159167,-21.3084818866879,
-15.217935174383));
#60638=CARTESIAN_POINT('Ctrl Pts',(-19.8168362586923,-21.2717124039116,
-15.2222513371219));
#60639=CARTESIAN_POINT('Ctrl Pts',(-19.8930399886395,-21.2361406831693,
-15.2264269013136));
#60640=CARTESIAN_POINT('Ctrl Pts',(-19.9674341519885,-21.1968356830556,
-15.2306024655052));
#60641=CARTESIAN_POINT('Ctrl Pts',(-20.0396421490702,-21.1540214755018,
-15.2347780296969));
#60642=CARTESIAN_POINT('Ctrl Pts',(-20.1154972004263,-21.1090448241057,
-15.2391644917094));
#60643=CARTESIAN_POINT('Ctrl Pts',(-20.188938948885,-21.0601954720668,-15.243550953722));
#60644=CARTESIAN_POINT('Ctrl Pts',(-20.259567662025,-21.0077828943212,-15.2479374157345));
#60645=CARTESIAN_POINT('Ctrl Pts',(-20.330196375165,-20.9553703165755,-15.252323877747));
#60646=CARTESIAN_POINT('Ctrl Pts',(-20.398011653933,-20.899394941135,-15.2567103397596));
#60647=CARTESIAN_POINT('Ctrl Pts',(-20.4626578964185,-20.8402112903883,
-15.2610968017721));
#60648=CARTESIAN_POINT('Ctrl Pts',(-20.5234100187943,-20.7845927075509,
-15.2652190348167));
#60649=CARTESIAN_POINT('Ctrl Pts',(-20.5816044022752,-20.7259204795934,
-15.2693412678613));
#60650=CARTESIAN_POINT('Ctrl Pts',(-20.6369112461382,-20.6644627847987,
-15.2734635009059));
#60651=CARTESIAN_POINT('Ctrl Pts',(-20.6921256485478,-20.6031078121671,
-15.2775788439313));
#60652=CARTESIAN_POINT('Ctrl Pts',(-20.7444617859852,-20.538976972769,-15.2816941869567));
#60653=CARTESIAN_POINT('Ctrl Pts',(-20.7936245240703,-20.4723771965695,
-15.2858095299821));
#60654=CARTESIAN_POINT('Ctrl Pts',(-20.8427410076358,-20.4058400804406,
-15.2899210011074));
#60655=CARTESIAN_POINT('Ctrl Pts',(-20.888689733586,-20.3368390147958,-15.2940324722326));
#60656=CARTESIAN_POINT('Ctrl Pts',(-20.9312146121388,-20.26571532236,-15.2981439433578));
#60657=CARTESIAN_POINT('Ctrl Pts',(-20.9737131282065,-20.1946357216972,
-15.3022528656552));
#60658=CARTESIAN_POINT('Ctrl Pts',(-21.0127917657816,-20.1214365120737,
-15.3063617879525));
#60659=CARTESIAN_POINT('Ctrl Pts',(-21.0482376124058,-20.0464881330222,
-15.3104707102499));
#60660=CARTESIAN_POINT('Ctrl Pts',(-21.0836728562216,-19.9715621730513,
-15.3145784034578));
#60661=CARTESIAN_POINT('Ctrl Pts',(-21.1154772648505,-19.8948885121031,
-15.3186860966657));
#60662=CARTESIAN_POINT('Ctrl Pts',(-21.1434845038947,-19.8168609284106,
-15.3227937898736));
#60663=CARTESIAN_POINT('Ctrl Pts',(-21.1715053065238,-19.7387955568538,
-15.3269034723903));
#60664=CARTESIAN_POINT('Ctrl Pts',(-21.1957251016683,-19.6593753990475,
-15.3310131549069));
#60665=CARTESIAN_POINT('Ctrl Pts',(-21.2160265895469,-19.5790119686115,
-15.3351228374236));
#60666=CARTESIAN_POINT('Ctrl Pts',(-21.2363332616042,-19.4986280166064,
-15.3392335693869));
#60667=CARTESIAN_POINT('Ctrl Pts',(-21.2527195357624,-19.4173007774455,
-15.3433443013502));
#60668=CARTESIAN_POINT('Ctrl Pts',(-21.265119175788,-19.3354523672614,-15.3474550333135));
#60669=CARTESIAN_POINT('Ctrl Pts',(-21.277533866187,-19.2535046115213,-15.3515707547806));
#60670=CARTESIAN_POINT('Ctrl Pts',(-21.2859522113271,-19.1710348943524,
-15.3556864762477));
#60671=CARTESIAN_POINT('Ctrl Pts',(-21.2903598951029,-19.0884700945603,
-15.3598021977147));
#60672=CARTESIAN_POINT('Ctrl Pts',(-21.2928257992759,-19.0422787399392,
-15.362104761886));
#60673=CARTESIAN_POINT('Ctrl Pts',(-21.294037342402,-18.9960576424384,-15.3644073260573));
#60674=CARTESIAN_POINT('Ctrl Pts',(-21.2939991231355,-18.9498811452879,
-15.3667098902285));
#60675=CARTESIAN_POINT('Origin',(-18.734,-18.952,1.76670989022851));
#60676=CARTESIAN_POINT('',(-17.1770150863476,-16.9251769922837,-14.0501277838374));
#60677=CARTESIAN_POINT('',(-17.17189441536,-16.9185281387053,-14.1167030432336));
#60678=CARTESIAN_POINT('',(-17.1744641548914,-16.9218650419685,1.76670989022851));
#60679=CARTESIAN_POINT('',(-21.2941233742573,-18.953130183291,-14.6332901097715));
#60680=CARTESIAN_POINT('Ctrl Pts',(-17.17189441536,-16.9185281387053,-14.1167030432336));
#60681=CARTESIAN_POINT('Ctrl Pts',(-16.5081486518363,-17.4296845150534,
-14.1585606262999));
#60682=CARTESIAN_POINT('Ctrl Pts',(-15.7210164188585,-19.1757114375145,
-14.2428101449267));
#60683=CARTESIAN_POINT('Ctrl Pts',(-17.2790525445471,-21.6065091564228,
-14.369451599114));
#60684=CARTESIAN_POINT('Ctrl Pts',(-20.1784866529944,-21.6122160192327,
-14.4966274057954));
#60685=CARTESIAN_POINT('Ctrl Pts',(-21.2671017221445,-19.9284206152422,
-14.5845735760146));
#60686=CARTESIAN_POINT('Ctrl Pts',(-21.2979708163172,-19.0164624131716,
-14.6301278106733));
#60687=CARTESIAN_POINT('Ctrl Pts',(-21.2976210374783,-18.9531317273574,
-14.6332901097715));
#60688=CARTESIAN_POINT('Ctrl Pts',(-21.2939997505486,-18.9531301287165,
-14.6332901097715));
#60689=CARTESIAN_POINT('Ctrl Pts',(-21.2940362985033,-18.8703406609988,
-14.6374299052976));
#60690=CARTESIAN_POINT('Ctrl Pts',(-21.2900525381051,-18.7873874928942,
-14.6415697008237));
#60691=CARTESIAN_POINT('Ctrl Pts',(-21.2820270867845,-18.7046986352398,
-14.6457094963498));
#60692=CARTESIAN_POINT('Ctrl Pts',(-21.2740124509524,-18.6221212131097,
-14.6498437128863));
#60693=CARTESIAN_POINT('Ctrl Pts',(-21.2619669829652,-18.5398078587026,
-14.6539779294227));
#60694=CARTESIAN_POINT('Ctrl Pts',(-21.2459213201025,-18.4581869973214,
-14.6581121459591));
#60695=CARTESIAN_POINT('Ctrl Pts',(-21.2298921267196,-18.3766499126674,
-14.6622421190812));
#60696=CARTESIAN_POINT('Ctrl Pts',(-21.2098709847548,-18.2958043686398,
-14.6663720922033));
#60697=CARTESIAN_POINT('Ctrl Pts',(-21.1859402178852,-18.2160725797221,
-14.6705020653254));
#60698=CARTESIAN_POINT('Ctrl Pts',(-21.1620224032905,-18.1363839447932,
-14.6746298031432));
#60699=CARTESIAN_POINT('Ctrl Pts',(-21.1341992976673,-18.0578083185522,
-14.6787575409609));
#60700=CARTESIAN_POINT('Ctrl Pts',(-21.1026037847562,-17.9807553805356,
-14.6828852787787));
#60701=CARTESIAN_POINT('Ctrl Pts',(-21.0710154147149,-17.9037198620526,
-14.6870120834293));
#60702=CARTESIAN_POINT('Ctrl Pts',(-21.0356565094079,-17.8282067834225,
-14.69113888808));
#60703=CARTESIAN_POINT('Ctrl Pts',(-20.9967085276618,-17.7546069488901,
-14.6952656927306));
#60704=CARTESIAN_POINT('Ctrl Pts',(-20.9577570758465,-17.6810005569824,
-14.6993928650588));
#60705=CARTESIAN_POINT('Ctrl Pts',(-20.9152161348637,-17.6093081624228,
-14.703520037387));
#60706=CARTESIAN_POINT('Ctrl Pts',(-20.8693129406038,-17.5398956675621,
-14.7076472097152));
#60707=CARTESIAN_POINT('Ctrl Pts',(-20.8233622278895,-17.4704113176916,
-14.7117786544444));
#60708=CARTESIAN_POINT('Ctrl Pts',(-20.7740425759674,-17.4032119705945,
-14.7159100991735));
#60709=CARTESIAN_POINT('Ctrl Pts',(-20.7216239583869,-17.3386336435743,
-14.7200415439027));
#60710=CARTESIAN_POINT('Ctrl Pts',(-20.6691749218115,-17.2740178411706,
-14.7241753861463));
#60711=CARTESIAN_POINT('Ctrl Pts',(-20.6136236562292,-17.2120264344647,
-14.7283092283899));
#60712=CARTESIAN_POINT('Ctrl Pts',(-20.5552780488236,-17.1529596255578,
-14.7324430706336));
#60713=CARTESIAN_POINT('Ctrl Pts',(-20.4968364594113,-17.0937956482246,
-14.7365837132944));
#60714=CARTESIAN_POINT('Ctrl Pts',(-20.4355917013472,-17.0375661867587,
-14.7407243559553));
#60715=CARTESIAN_POINT('Ctrl Pts',(-20.3718854170603,-16.9845317383548,
-14.7448649986162));
#60716=CARTESIAN_POINT('Ctrl Pts',(-20.3405294527256,-16.9584284066148,
-14.7469030054636));
#60717=CARTESIAN_POINT('Ctrl Pts',(-20.3085776248464,-16.9330984310457,
-14.7489410123109));
#60718=CARTESIAN_POINT('Ctrl Pts',(-20.2760730898183,-16.9085689182999,
-14.7509790191583));
#60719=CARTESIAN_POINT('Ctrl Pts',(-20.2093316088542,-16.8582025307612,
-14.7551636535514));
#60720=CARTESIAN_POINT('Ctrl Pts',(-20.1399957688999,-16.811015665153,-14.7593482879444));
#60721=CARTESIAN_POINT('Ctrl Pts',(-20.0684012262925,-16.767286433587,-14.7635329223375));
#60722=CARTESIAN_POINT('Ctrl Pts',(-19.9969085896549,-16.7236194451695,
-14.7677116004214));
#60723=CARTESIAN_POINT('Ctrl Pts',(-19.9231640255692,-16.6834005528598,
-14.7718902785053));
#60724=CARTESIAN_POINT('Ctrl Pts',(-19.8475347050067,-16.6468664982814,
-14.7760689565893));
#60725=CARTESIAN_POINT('Ctrl Pts',(-19.7705497832269,-16.6096775970311,
-14.7803225344747));
#60726=CARTESIAN_POINT('Ctrl Pts',(-19.6916122567006,-16.5763072247155,
-14.7845761123601));
#60727=CARTESIAN_POINT('Ctrl Pts',(-19.6111386006651,-16.5469578225688,
-14.7888296902456));
#60728=CARTESIAN_POINT('Ctrl Pts',(-19.5322250834833,-16.5181774158532,
-14.7930008042235));
#60729=CARTESIAN_POINT('Ctrl Pts',(-19.4518349191003,-16.4932636267838,
-14.7971719182015));
#60730=CARTESIAN_POINT('Ctrl Pts',(-19.3703822558338,-16.4723593759458,
-14.8013430321794));
#60731=CARTESIAN_POINT('Ctrl Pts',(-19.288956924795,-16.4514621397311,-14.8055127464998));
#60732=CARTESIAN_POINT('Ctrl Pts',(-19.2064702481718,-16.4345718839471,
-14.8096824608202));
#60733=CARTESIAN_POINT('Ctrl Pts',(-19.1233507011893,-16.4217814261445,
-14.8138521751405));
#60734=CARTESIAN_POINT('Ctrl Pts',(-19.0402341119571,-16.4089914234813,
-14.8180217410846));
#60735=CARTESIAN_POINT('Ctrl Pts',(-18.9564851519522,-16.4003009978601,
-14.8221913070286));
#60736=CARTESIAN_POINT('Ctrl Pts',(-18.87254027672,-16.3957514612764,-14.8263608729727));
#60737=CARTESIAN_POINT('Ctrl Pts',(-18.7856440032318,-16.3910419685989,
-14.8306770357116));
#60738=CARTESIAN_POINT('Ctrl Pts',(-18.6985383080789,-16.3907699986349,
-14.8349931984505));
#60739=CARTESIAN_POINT('Ctrl Pts',(-18.611708547389,-16.3949226056652,-14.8393093611894));
#60740=CARTESIAN_POINT('Ctrl Pts',(-18.5277072570206,-16.3989399419582,
-14.8434849253811));
#60741=CARTESIAN_POINT('Ctrl Pts',(-18.4439646643006,-16.4070979281598,
-14.8476604895728));
#60742=CARTESIAN_POINT('Ctrl Pts',(-18.3609142114861,-16.4193320402372,
-14.8518360537644));
#60743=CARTESIAN_POINT('Ctrl Pts',(-18.2736690777338,-16.4321840682319,
-14.856222515777));
#60744=CARTESIAN_POINT('Ctrl Pts',(-18.1871884138653,-16.4495346990029,
-14.8606089777895));
#60745=CARTESIAN_POINT('Ctrl Pts',(-18.1019594530764,-16.471249156597,-14.864995439802));
#60746=CARTESIAN_POINT('Ctrl Pts',(-18.0167304922876,-16.4929636141912,
-14.8693819018146));
#60747=CARTESIAN_POINT('Ctrl Pts',(-17.932753766134,-16.5190416538915,-14.8737683638271));
#60748=CARTESIAN_POINT('Ctrl Pts',(-17.8504927560606,-16.549290082031,-14.8781548258397));
#60749=CARTESIAN_POINT('Ctrl Pts',(-17.7720269461594,-16.5781429664058,
-14.8823389137096));
#60750=CARTESIAN_POINT('Ctrl Pts',(-17.6948300019267,-16.6108972906705,
-14.8865230015795));
#60751=CARTESIAN_POINT('Ctrl Pts',(-17.6193172941295,-16.6474214126584,
-14.8907070894494));
#60752=CARTESIAN_POINT('Ctrl Pts',(-17.5409561860664,-16.6853232539975,
-14.8950490044897));
#60753=CARTESIAN_POINT('Ctrl Pts',(-17.4644093908721,-16.7272848596456,
-14.89939091953));
#60754=CARTESIAN_POINT('Ctrl Pts',(-17.3901227433324,-16.7731025909852,
-14.9037328345703));
#60755=CARTESIAN_POINT('Ctrl Pts',(-17.3158360957927,-16.8189203223247,
-14.9080747496106));
#60756=CARTESIAN_POINT('Ctrl Pts',(-17.2438101074633,-16.8685939536001,
-14.9124166646509));
#60757=CARTESIAN_POINT('Ctrl Pts',(-17.1744641548914,-16.9218650419685,
-14.9167585796912));
#60758=CARTESIAN_POINT('',(-21.2936354977614,-18.9514398261094,-14.566709915054));
#60759=CARTESIAN_POINT('Ctrl Pts',(-21.2939999386838,-18.9514396975034,
-14.566709917474));
#60760=CARTESIAN_POINT('Ctrl Pts',(-21.2939802627005,-18.8615409084184,
-14.571157199273));
#60761=CARTESIAN_POINT('Ctrl Pts',(-21.2892209204008,-18.7717655181781,
-14.575604481072));
#60762=CARTESIAN_POINT('Ctrl Pts',(-21.2797861099468,-18.6826060832129,
-14.5800517628709));
#60763=CARTESIAN_POINT('Ctrl Pts',(-21.2703167670437,-18.5931203148612,
-14.5845153222128));
#60764=CARTESIAN_POINT('Ctrl Pts',(-21.2561377674616,-18.5042553694628,
-14.5889788815547));
#60765=CARTESIAN_POINT('Ctrl Pts',(-21.2373647797459,-18.4164957707656,
-14.5934424408966));
#60766=CARTESIAN_POINT('Ctrl Pts',(-21.2185553401018,-18.3285657673013,
-14.5979146672311));
#60767=CARTESIAN_POINT('Ctrl Pts',(-21.1951342035189,-18.2417457397356,
-14.6023868935656));
#60768=CARTESIAN_POINT('Ctrl Pts',(-21.1672666877164,-18.1565044145631,
-14.6068591199));
#60769=CARTESIAN_POINT('Ctrl Pts',(-21.139316159677,-18.0710091710603,-14.6113446681795));
#60770=CARTESIAN_POINT('Ctrl Pts',(-21.1068928974786,-17.9871023685111,
-14.6158302164589));
#60771=CARTESIAN_POINT('Ctrl Pts',(-21.0702104967804,-17.9052333045357,
-14.6203157647383));
#60772=CARTESIAN_POINT('Ctrl Pts',(-21.0568477853901,-17.875409938211,-14.6219497659472));
#60773=CARTESIAN_POINT('Ctrl Pts',(-21.0429203172351,-17.8458567318452,
-14.6235837671561));
#60774=CARTESIAN_POINT('Ctrl Pts',(-21.0284398795323,-17.8165945044999,
-14.625217768365));
#60775=CARTESIAN_POINT('Ctrl Pts',(-20.9913558570061,-17.7416547050056,
-14.629402402758));
#60776=CARTESIAN_POINT('Ctrl Pts',(-20.9505274948144,-17.6683941847451,
-14.6335870371511));
#60777=CARTESIAN_POINT('Ctrl Pts',(-20.9061301751471,-17.5972120083883,
-14.6377716715441));
#60778=CARTESIAN_POINT('Ctrl Pts',(-20.8617960495691,-17.526131151049,-14.641950349628));
#60779=CARTESIAN_POINT('Ctrl Pts',(-20.8139032983065,-17.4571231485616,
-14.646129027712));
#60780=CARTESIAN_POINT('Ctrl Pts',(-20.7626740190629,-17.3905642106128,
-14.6503077057959));
#60781=CARTESIAN_POINT('Ctrl Pts',(-20.7105264918066,-17.3228122515362,
-14.6545612836814));
#60782=CARTESIAN_POINT('Ctrl Pts',(-20.6549218593555,-17.2575984516732,
-14.6588148615668));
#60783=CARTESIAN_POINT('Ctrl Pts',(-20.5961416680529,-17.1952904599504,
-14.6630684394522));
#60784=CARTESIAN_POINT('Ctrl Pts',(-20.5385010454588,-17.1341904302312,
-14.6672395534302));
#60785=CARTESIAN_POINT('Ctrl Pts',(-20.4778072242624,-17.0758848946115,
-14.6714106674081));
#60786=CARTESIAN_POINT('Ctrl Pts',(-20.4143663508876,-17.0206872529793,
-14.6755817813861));
#60787=CARTESIAN_POINT('Ctrl Pts',(-20.3509467657106,-16.9655081334487,
-14.6797514957065));
#60788=CARTESIAN_POINT('Ctrl Pts',(-20.2847823058332,-16.9134351384329,
-14.6839212100268));
#60789=CARTESIAN_POINT('Ctrl Pts',(-20.2162143833073,-16.8647433023423,
-14.6880909243472));
#60790=CARTESIAN_POINT('Ctrl Pts',(-20.1476489007224,-16.8160531989162,
-14.6922604902913));
#60791=CARTESIAN_POINT('Ctrl Pts',(-20.0766805011099,-16.7707442808556,
-14.6964300562353));
#60792=CARTESIAN_POINT('Ctrl Pts',(-20.003680817563,-16.729049118511,-14.7005996221794));
#60793=CARTESIAN_POINT('Ctrl Pts',(-19.9281145551974,-16.685888005695,-14.7049157849183));
#60794=CARTESIAN_POINT('Ctrl Pts',(-19.850371969323,-16.6465997576133,-14.7092319476572));
#60795=CARTESIAN_POINT('Ctrl Pts',(-19.7708927266887,-16.6113903628883,
-14.7135481103961));
#60796=CARTESIAN_POINT('Ctrl Pts',(-19.6940025120234,-16.5773279104931,
-14.7177236745878));
#60797=CARTESIAN_POINT('Ctrl Pts',(-19.6154875027973,-16.5470827802972,
-14.7218992387795));
#60798=CARTESIAN_POINT('Ctrl Pts',(-19.5357640795052,-16.5207915842497,
-14.7260748029712));
#60799=CARTESIAN_POINT('Ctrl Pts',(-19.4520140156271,-16.4931724823912,
-14.7304612649837));
#60800=CARTESIAN_POINT('Ctrl Pts',(-19.3669308187544,-16.4699173921691,
-14.7348477269962));
#60801=CARTESIAN_POINT('Ctrl Pts',(-19.2810104439706,-16.4511242385542,
-14.7392341890088));
#60802=CARTESIAN_POINT('Ctrl Pts',(-19.1950900691869,-16.4323310849393,
-14.7436206510213));
#60803=CARTESIAN_POINT('Ctrl Pts',(-19.1083331013483,-16.4179998874471,
-14.7480071130339));
#60804=CARTESIAN_POINT('Ctrl Pts',(-19.021240449396,-16.4081657042506,-14.7523935750464));
#60805=CARTESIAN_POINT('Ctrl Pts',(-18.9381783893877,-16.3987866407305,
-14.7565770344169));
#60806=CARTESIAN_POINT('Ctrl Pts',(-18.854501943096,-16.3934626556781,-14.7607604937874));
#60807=CARTESIAN_POINT('Ctrl Pts',(-18.7706412277849,-16.3922622360042,
-14.7649439531578));
#60808=CARTESIAN_POINT('Ctrl Pts',(-18.6868897531745,-16.3910633800504,
-14.7691219629679));
#60809=CARTESIAN_POINT('Ctrl Pts',(-18.6029549415358,-16.3939774328896,
-14.773299972778));
#60810=CARTESIAN_POINT('Ctrl Pts',(-18.5192731319703,-16.4010212913185,
-14.7774779825881));
#60811=CARTESIAN_POINT('Ctrl Pts',(-18.4356752189539,-16.4080580878134,
-14.781651803667));
#60812=CARTESIAN_POINT('Ctrl Pts',(-18.3523302600701,-16.4192164297761,
-14.7858256247459));
#60813=CARTESIAN_POINT('Ctrl Pts',(-18.2696743384303,-16.4344611859977,
-14.7899994458248));
#60814=CARTESIAN_POINT('Ctrl Pts',(-18.1870764857767,-16.4496952321877,
-14.7941703346327));
#60815=CARTESIAN_POINT('Ctrl Pts',(-18.1051671597325,-16.4690099061388,
-14.7983412234407));
#60816=CARTESIAN_POINT('Ctrl Pts',(-18.0243757041687,-16.4923184436261,
-14.8025121122486));
#60817=CARTESIAN_POINT('Ctrl Pts',(-17.9435959999426,-16.5156235908231,
-14.8066823943894));
#60818=CARTESIAN_POINT('Ctrl Pts',(-17.8639342884434,-16.5429213326383,
-14.8108526765302));
#60819=CARTESIAN_POINT('Ctrl Pts',(-17.7858071130399,-16.5740743810795,
-14.8150229586709));
#60820=CARTESIAN_POINT('Ctrl Pts',(-17.7076898405936,-16.6052234807372,
-14.8191927122104));
#60821=CARTESIAN_POINT('Ctrl Pts',(-17.631107142899,-16.6402267397327,-14.82336246575));
#60822=CARTESIAN_POINT('Ctrl Pts',(-17.5564562226973,-16.6788984508967,
-14.8275322192895));
#60823=CARTESIAN_POINT('Ctrl Pts',(-17.4817531859644,-16.7175971601933,
-14.831704883886));
#60824=CARTESIAN_POINT('Ctrl Pts',(-17.4089850280066,-16.7599692220366,
-14.8358775484826));
#60825=CARTESIAN_POINT('Ctrl Pts',(-17.3385243273809,-16.8057829450104,
-14.8400502130792));
#60826=CARTESIAN_POINT('Ctrl Pts',(-17.2823110146712,-16.8423329808893,
-14.8433791510222));
#60827=CARTESIAN_POINT('Ctrl Pts',(-17.2275659250877,-16.8810726238427,
-14.8467080889651));
#60828=CARTESIAN_POINT('Ctrl Pts',(-17.1744641548915,-16.9218650419685,
-14.8500370269081));
#60829=CARTESIAN_POINT('Ctrl Pts',(-17.1770150863476,-16.9251769922837,
-14.0501277838374));
#60830=CARTESIAN_POINT('Ctrl Pts',(-16.8231471804876,-17.1976900874761,
-14.0722567031047));
#60831=CARTESIAN_POINT('Ctrl Pts',(-15.9876142224497,-18.2487089372057,
-14.1367775579324));
#60832=CARTESIAN_POINT('Ctrl Pts',(-16.2435266831926,-20.6727072634931,
-14.2436903483206));
#60833=CARTESIAN_POINT('Ctrl Pts',(-18.8327965299441,-21.9774801394222,
-14.3708661550021));
#60834=CARTESIAN_POINT('Ctrl Pts',(-20.9482575115022,-20.7321304478324,
-14.478539335638));
#60835=CARTESIAN_POINT('Ctrl Pts',(-21.2889974874197,-19.4133916920799,
-14.5438205807135));
#60836=CARTESIAN_POINT('Ctrl Pts',(-21.2898969963344,-18.9514411453738,
-14.5667098902285));
#60837=CARTESIAN_POINT('Origin',(-18.734,-18.952,1.76670989022851));
#60838=CARTESIAN_POINT('',(-17.1744641548914,-16.9218650419685,-13.250188010165));
#60839=CARTESIAN_POINT('',(-17.1744641548914,-16.9218650419685,-13.3166223748392));
#60840=CARTESIAN_POINT('',(-17.1744641548914,-16.9218650419685,1.76670989022851));
#60841=CARTESIAN_POINT('',(-21.2939989424941,-18.949673107456,-13.8332901097715));
#60842=CARTESIAN_POINT('Ctrl Pts',(-17.1744641548914,-16.9218650419685,
-13.3166223748392));
#60843=CARTESIAN_POINT('Ctrl Pts',(-17.1077897102854,-16.9730838961163,
-13.3207986479985));
#60844=CARTESIAN_POINT('Ctrl Pts',(-17.0436958183771,-17.027548772347,-13.3249749211578));
#60845=CARTESIAN_POINT('Ctrl Pts',(-16.9824997154987,-17.0849577526495,
-13.329151194317));
#60846=CARTESIAN_POINT('Ctrl Pts',(-16.9211959283922,-17.1424677531384,
-13.3333348162899));
#60847=CARTESIAN_POINT('Ctrl Pts',(-16.8628004366934,-17.202931875454,-13.3375184382627));
#60848=CARTESIAN_POINT('Ctrl Pts',(-16.807592344652,-17.2660125903742,-13.3417020602355));
#60849=CARTESIAN_POINT('Ctrl Pts',(-16.762095721873,-17.3179969894946,-13.3451497553778));
#60850=CARTESIAN_POINT('Ctrl Pts',(-16.7187630874481,-17.3717576702114,
-13.3485974505202));
#60851=CARTESIAN_POINT('Ctrl Pts',(-16.677728404917,-17.4270911085396,-13.3520451456625));
#60852=CARTESIAN_POINT('Ctrl Pts',(-16.6279226254792,-17.4942519796595,
-13.3562297800555));
#60853=CARTESIAN_POINT('Ctrl Pts',(-16.5813179797007,-17.5639804959206,
-13.3604144144486));
#60854=CARTESIAN_POINT('Ctrl Pts',(-16.5381897594127,-17.6359386840531,
-13.3645990488416));
#60855=CARTESIAN_POINT('Ctrl Pts',(-16.495122926808,-17.7077944486115,-13.3687777269256));
#60856=CARTESIAN_POINT('Ctrl Pts',(-16.4555229253634,-17.7818731899371,
-13.3729564050095));
#60857=CARTESIAN_POINT('Ctrl Pts',(-16.4196234139921,-17.8578057676361,
-13.3771350830935));
#60858=CARTESIAN_POINT('Ctrl Pts',(-16.3830804296801,-17.9350993822185,
-13.3813886609789));
#60859=CARTESIAN_POINT('Ctrl Pts',(-16.350372190068,-18.0143135596368,-13.3856422388643));
#60860=CARTESIAN_POINT('Ctrl Pts',(-16.3216976420462,-18.0950301441646,
-13.3898958167498));
#60861=CARTESIAN_POINT('Ctrl Pts',(-16.2935790060915,-18.1741818801959,
-13.3940669307277));
#60862=CARTESIAN_POINT('Ctrl Pts',(-16.2693392165557,-18.2547778355446,
-13.3982380447057));
#60863=CARTESIAN_POINT('Ctrl Pts',(-16.2491177212505,-18.3364026797033,
-13.4024091586836));
#60864=CARTESIAN_POINT('Ctrl Pts',(-16.2289030114633,-18.4180001338573,
-13.406578873004));
#60865=CARTESIAN_POINT('Ctrl Pts',(-16.2127040285388,-18.5006253449796,
-13.4107485873244));
#60866=CARTESIAN_POINT('Ctrl Pts',(-16.2006099990479,-18.5838490756822,
-13.4149183016447));
#60867=CARTESIAN_POINT('Ctrl Pts',(-16.1885163999146,-18.6670698449272,
-13.4190878675888));
#60868=CARTESIAN_POINT('Ctrl Pts',(-16.1805275291,-18.7508886360331,-13.4232574335328));
#60869=CARTESIAN_POINT('Ctrl Pts',(-16.1766810426044,-18.8348686628402,
-13.4274269994769));
#60870=CARTESIAN_POINT('Ctrl Pts',(-16.1726993183887,-18.9218013237893,
-13.4317431622158));
#60871=CARTESIAN_POINT('Ctrl Pts',(-16.1731567148617,-19.0089062426184,
-13.4360593249547));
#60872=CARTESIAN_POINT('Ctrl Pts',(-16.1780362227548,-19.095698188612,-13.4403754876936));
#60873=CARTESIAN_POINT('Ctrl Pts',(-16.1827567811915,-19.1796628960938,
-13.4445510518853));
#60874=CARTESIAN_POINT('Ctrl Pts',(-16.1916156782437,-19.2633342443402,
-13.448726616077));
#60875=CARTESIAN_POINT('Ctrl Pts',(-16.2045447628248,-19.346279346564,-13.4529021802687));
#60876=CARTESIAN_POINT('Ctrl Pts',(-16.2181268647321,-19.4334138087178,
-13.4572886422812));
#60877=CARTESIAN_POINT('Ctrl Pts',(-16.236201010622,-19.5197461599059,-13.4616751042937));
#60878=CARTESIAN_POINT('Ctrl Pts',(-16.2586283495454,-19.6047903125243,
-13.4660615663063));
#60879=CARTESIAN_POINT('Ctrl Pts',(-16.2810556884688,-19.6898344651427,
-13.4704480283188));
#60880=CARTESIAN_POINT('Ctrl Pts',(-16.3078359712666,-19.7735898897036,
-13.4748344903314));
#60881=CARTESIAN_POINT('Ctrl Pts',(-16.3387721302028,-19.8555947386669,
-13.4792209523439));
#60882=CARTESIAN_POINT('Ctrl Pts',(-16.3682848706079,-19.9338264229691,
-13.4834055867369));
#60883=CARTESIAN_POINT('Ctrl Pts',(-16.4016893071736,-20.0107562780699,
-13.48759022113));
#60884=CARTESIAN_POINT('Ctrl Pts',(-16.4388502681124,-20.0859698885844,
-13.491774855523));
#60885=CARTESIAN_POINT('Ctrl Pts',(-16.4759583350229,-20.1610764418341,
-13.495953533607));
#60886=CARTESIAN_POINT('Ctrl Pts',(-16.5168121035543,-20.2344711938782,
-13.5001322116909));
#60887=CARTESIAN_POINT('Ctrl Pts',(-16.5612276601911,-20.3057578658539,
-13.5043108897749));
#60888=CARTESIAN_POINT('Ctrl Pts',(-16.6064393337596,-20.3783223001918,
-13.5085644676603));
#60889=CARTESIAN_POINT('Ctrl Pts',(-16.6553415713119,-20.4487018853352,
-13.5128180455458));
#60890=CARTESIAN_POINT('Ctrl Pts',(-16.707690456235,-20.5165029986698,-13.5170716234312));
#60891=CARTESIAN_POINT('Ctrl Pts',(-16.7590244558735,-20.5829896551195,
-13.5212427374092));
#60892=CARTESIAN_POINT('Ctrl Pts',(-16.8136723614036,-20.6469965440965,
-13.5254138513871));
#60893=CARTESIAN_POINT('Ctrl Pts',(-16.8713604260518,-20.7081816015327,
-13.5295849653651));
#60894=CARTESIAN_POINT('Ctrl Pts',(-16.9290291329127,-20.769346127732,-13.5337546796854));
#60895=CARTESIAN_POINT('Ctrl Pts',(-16.9897356575244,-20.8276903684962,
-13.5379243940058));
#60896=CARTESIAN_POINT('Ctrl Pts',(-17.0531673758224,-20.8829069603428,
-13.5420941083262));
#60897=CARTESIAN_POINT('Ctrl Pts',(-17.1165968369475,-20.9381215873459,
-13.5462636742702));
#60898=CARTESIAN_POINT('Ctrl Pts',(-17.1827509514054,-20.9902084853113,
-13.5504332402143));
#60899=CARTESIAN_POINT('Ctrl Pts',(-17.251282833637,-21.0388995674379,-13.5546028061583));
#60900=CARTESIAN_POINT('Ctrl Pts',(-17.3222242123048,-21.0893025679452,
-13.5589189688972));
#60901=CARTESIAN_POINT('Ctrl Pts',(-17.3957132444234,-21.1360662103826,
-13.5632351316361));
#60902=CARTESIAN_POINT('Ctrl Pts',(-17.4713327209561,-21.1789421506703,
-13.5675512943751));
#60903=CARTESIAN_POINT('Ctrl Pts',(-17.5444889009946,-21.2204214117129,
-13.5717268585667));
#60904=CARTESIAN_POINT('Ctrl Pts',(-17.619638416544,-21.2582621950959,-13.5759024227584));
#60905=CARTESIAN_POINT('Ctrl Pts',(-17.6963803894315,-21.2922874916906,
-13.5800779869501));
#60906=CARTESIAN_POINT('Ctrl Pts',(-17.7769984169327,-21.3280313251289,
-13.5844644489626));
#60907=CARTESIAN_POINT('Ctrl Pts',(-17.8593734542579,-21.3595638930066,
-13.5888509109752));
#60908=CARTESIAN_POINT('Ctrl Pts',(-17.9430216212721,-21.3867388369977,
-13.5932373729877));
#60909=CARTESIAN_POINT('Ctrl Pts',(-18.0266697882863,-21.4139137809888,
-13.5976238350002));
#60910=CARTESIAN_POINT('Ctrl Pts',(-18.1115905049088,-21.4367310239951,
-13.6020102970128));
#60911=CARTESIAN_POINT('Ctrl Pts',(-18.1972887614197,-21.4551062794819,
-13.6063967590253));
#60912=CARTESIAN_POINT('Ctrl Pts',(-18.2790439141132,-21.4726360622251,
-13.6105813934184));
#60913=CARTESIAN_POINT('Ctrl Pts',(-18.3618109357871,-21.4861888889159,
-13.6147660278114));
#60914=CARTESIAN_POINT('Ctrl Pts',(-18.4451682027606,-21.4956541024486,
-13.6189506622044));
#60915=CARTESIAN_POINT('Ctrl Pts',(-18.5284068209818,-21.5051058434213,
-13.6231293402884));
#60916=CARTESIAN_POINT('Ctrl Pts',(-18.6122335625321,-21.5104814765753,
-13.6273080183723));
#60917=CARTESIAN_POINT('Ctrl Pts',(-18.6962156707026,-21.5117211458398,
-13.6314866964562));
#60918=CARTESIAN_POINT('Ctrl Pts',(-18.7817030978056,-21.512983035285,-13.6357402743417));
#60919=CARTESIAN_POINT('Ctrl Pts',(-18.8673510447832,-21.5099591270342,
-13.6399938522271));
#60920=CARTESIAN_POINT('Ctrl Pts',(-18.9526965098726,-21.5026414559027,
-13.6442474301125));
#60921=CARTESIAN_POINT('Ctrl Pts',(-19.0363873865832,-21.4954656521054,
-13.6484185440905));
#60922=CARTESIAN_POINT('Ctrl Pts',(-19.1197869256869,-21.4841611267898,
-13.6525896580684));
#60923=CARTESIAN_POINT('Ctrl Pts',(-19.2024593314988,-21.4687729048787,
-13.6567607720464));
#60924=CARTESIAN_POINT('Ctrl Pts',(-19.2851039957867,-21.4533898466341,
-13.6609304863668));
#60925=CARTESIAN_POINT('Ctrl Pts',(-19.3670215594753,-21.4339258973911,
-13.6651002006872));
#60926=CARTESIAN_POINT('Ctrl Pts',(-19.4477843610403,-21.4104775544906,
-13.6692699150075));
#60927=CARTESIAN_POINT('Ctrl Pts',(-19.5285442887181,-21.3870300459828,
-13.6734394809516));
#60928=CARTESIAN_POINT('Ctrl Pts',(-19.6081490944209,-21.3595985548019,
-13.6776090468956));
#60929=CARTESIAN_POINT('Ctrl Pts',(-19.6861855970008,-21.3283296465062,
-13.6817786128397));
#60930=CARTESIAN_POINT('Ctrl Pts',(-19.766965766743,-21.2959613619692,-13.6860947755786));
#60931=CARTESIAN_POINT('Ctrl Pts',(-19.8460648087822,-21.2594809885576,
-13.6904109383175));
#60932=CARTESIAN_POINT('Ctrl Pts',(-19.9230480777099,-21.2191049091064,
-13.6947271010565));
#60933=CARTESIAN_POINT('Ctrl Pts',(-19.9975236247494,-21.1800440761966,
-13.6989026652482));
#60934=CARTESIAN_POINT('Ctrl Pts',(-20.0700187425842,-21.1373377246263,
-13.7030782294398));
#60935=CARTESIAN_POINT('Ctrl Pts',(-20.1401676067978,-21.0912271178144,
-13.7072537936315));
#60936=CARTESIAN_POINT('Ctrl Pts',(-20.2138595233798,-21.04278757387,-13.7116402556441));
#60937=CARTESIAN_POINT('Ctrl Pts',(-20.2849614681661,-20.9905911845414,
-13.7160267176566));
#60938=CARTESIAN_POINT('Ctrl Pts',(-20.3530884618265,-20.9349655954605,
-13.7204131796692));
#60939=CARTESIAN_POINT('Ctrl Pts',(-20.4212154554869,-20.8793400063797,
-13.7247996416817));
#60940=CARTESIAN_POINT('Ctrl Pts',(-20.4863671192074,-20.8202856635708,
-13.7291861036942));
#60941=CARTESIAN_POINT('Ctrl Pts',(-20.548204641978,-20.7581731691688,-13.7335725657068));
#60942=CARTESIAN_POINT('Ctrl Pts',(-20.6067777194386,-20.6993396360183,
-13.7377274633762));
#60943=CARTESIAN_POINT('Ctrl Pts',(-20.6626103382647,-20.6375286216454,
-13.7418823610455));
#60944=CARTESIAN_POINT('Ctrl Pts',(-20.7153787245626,-20.5730300274365,
-13.7460372587149));
#60945=CARTESIAN_POINT('Ctrl Pts',(-20.7677053791601,-20.5090713601742,
-13.7501573751423));
#60946=CARTESIAN_POINT('Ctrl Pts',(-20.8170185699061,-20.4424702805591,
-13.7542774915697));
#60947=CARTESIAN_POINT('Ctrl Pts',(-20.8630375889924,-20.3735480803185,
-13.7583976079971));
#60948=CARTESIAN_POINT('Ctrl Pts',(-20.909012526032,-20.3046919012951,-13.7625137777266));
#60949=CARTESIAN_POINT('Ctrl Pts',(-20.9516992900879,-20.233519404422,-13.7666299474561));
#60950=CARTESIAN_POINT('Ctrl Pts',(-20.9908578231796,-20.1603843618457,
-13.7707461171856));
#60951=CARTESIAN_POINT('Ctrl Pts',(-21.0299913601116,-20.0872960037352,
-13.7748596594307));
#60952=CARTESIAN_POINT('Ctrl Pts',(-21.0656009133713,-20.0122480031423,
-13.7789732016758));
#60953=CARTESIAN_POINT('Ctrl Pts',(-21.0974909394085,-19.9356211564083,
-13.7830867439209));
#60954=CARTESIAN_POINT('Ctrl Pts',(-21.1299241917561,-19.8576890200775,
-13.7872703577418));
#60955=CARTESIAN_POINT('Ctrl Pts',(-21.158509766141,-19.7781241832438,-13.7914539715627));
#60956=CARTESIAN_POINT('Ctrl Pts',(-21.1830923574769,-19.6973500013741,
-13.7956375853835));
#60957=CARTESIAN_POINT('Ctrl Pts',(-21.2072638620763,-19.6179265800633,
-13.7997512379815));
#60958=CARTESIAN_POINT('Ctrl Pts',(-21.227565151866,-19.5373344318,-13.8038648905795));
#60959=CARTESIAN_POINT('Ctrl Pts',(-21.2438990336339,-19.4559909135726,
-13.8079785431775));
#60960=CARTESIAN_POINT('Ctrl Pts',(-21.260649602877,-19.372572271641,-13.8121971376098));
#60961=CARTESIAN_POINT('Ctrl Pts',(-21.2732274574716,-19.2883639128976,
-13.8164157320421));
#60962=CARTESIAN_POINT('Ctrl Pts',(-21.2815840465261,-19.2038243949373,
-13.8206343264745));
#60963=CARTESIAN_POINT('Ctrl Pts',(-21.2899406355806,-19.119284876977,-13.8248529209068));
#60964=CARTESIAN_POINT('Ctrl Pts',(-21.2940759677847,-19.0344147354448,
-13.8290715153392));
#60965=CARTESIAN_POINT('Ctrl Pts',(-21.2939989424941,-18.949673107456,-13.8332901097715));
#60966=CARTESIAN_POINT('Ctrl Pts',(-21.294449633852,-18.9496726978033,-13.8332901097715));
#60967=CARTESIAN_POINT('Ctrl Pts',(-21.2961551522482,-18.7657813487039,
-13.8424428639771));
#60968=CARTESIAN_POINT('Ctrl Pts',(-21.1940976782198,-17.7320561538789,
-13.8939875537431));
#60969=CARTESIAN_POINT('Ctrl Pts',(-19.7898862958127,-16.1150306505046,
-13.9879241790696));
#60970=CARTESIAN_POINT('Ctrl Pts',(-17.8646300934828,-16.3924604551013,
-14.0732424026848));
#60971=CARTESIAN_POINT('Ctrl Pts',(-17.1803677713987,-16.9120027336387,
-14.1161686907394));
#60972=CARTESIAN_POINT('Ctrl Pts',(-17.17189441536,-16.9185281387053,-14.1167030432336));
#60973=CARTESIAN_POINT('',(-21.2939989173812,-18.9543543592142,-13.7667098774877));
#60974=CARTESIAN_POINT('Ctrl Pts',(-21.2935815865034,-18.9543537192076,
-13.7667098902285));
#60975=CARTESIAN_POINT('Ctrl Pts',(-21.2877697346816,-18.3145386563719,
-13.7985275695778));
#60976=CARTESIAN_POINT('Ctrl Pts',(-20.7208249375185,-16.8130884735802,
-13.8727371844876));
#60977=CARTESIAN_POINT('Ctrl Pts',(-18.6774626831344,-16.1321013561092,
-13.9672098156905));
#60978=CARTESIAN_POINT('Ctrl Pts',(-17.5010449702959,-16.675642108935,-14.0298647675442));
#60979=CARTESIAN_POINT('Ctrl Pts',(-17.1770150863476,-16.9251769922837,
-14.0501277838374));
#60980=CARTESIAN_POINT('Ctrl Pts',(-17.1744641548914,-16.9218650419685,
-13.250188010165));
#60981=CARTESIAN_POINT('Ctrl Pts',(-17.1058905228881,-16.9745428389373,
-13.2544909973061));
#60982=CARTESIAN_POINT('Ctrl Pts',(-17.0399075290738,-17.0307614250666,
-13.2587939844472));
#60983=CARTESIAN_POINT('Ctrl Pts',(-16.9768962778943,-17.0902302747756,
-13.2630969715882));
#60984=CARTESIAN_POINT('Ctrl Pts',(-16.915813603391,-17.1478789696017,-13.2672682577952));
#60985=CARTESIAN_POINT('Ctrl Pts',(-16.8575237492257,-17.2085815017709,
-13.2714395440022));
#60986=CARTESIAN_POINT('Ctrl Pts',(-16.8023405437521,-17.2720322190328,
-13.2756108302092));
#60987=CARTESIAN_POINT('Ctrl Pts',(-16.7471772277534,-17.3354600669916,
-13.2797806129752));
#60988=CARTESIAN_POINT('Ctrl Pts',(-16.695118638371,-17.4016337861567,-13.2839503957412));
#60989=CARTESIAN_POINT('Ctrl Pts',(-16.6464403094113,-17.4702123842368,
-13.2881201785072));
#60990=CARTESIAN_POINT('Ctrl Pts',(-16.5977649230779,-17.5387868367106,
-13.292289709208));
#60991=CARTESIAN_POINT('Ctrl Pts',(-16.5524696567119,-17.6097655036099,
-13.2964592399087));
#60992=CARTESIAN_POINT('Ctrl Pts',(-16.5107876396202,-17.6827770878784,
-13.3006287706095));
#60993=CARTESIAN_POINT('Ctrl Pts',(-16.4690956388469,-17.75580615989,-13.3047992999968));
#60994=CARTESIAN_POINT('Ctrl Pts',(-16.431018832745,-17.8308687160974,-13.3089698293841));
#60995=CARTESIAN_POINT('Ctrl Pts',(-16.3967445142583,-17.9075686741723,
-13.3131403587714));
#60996=CARTESIAN_POINT('Ctrl Pts',(-16.3624311151704,-17.9843560878291,
-13.3173156435208));
#60997=CARTESIAN_POINT('Ctrl Pts',(-16.3319290415391,-18.0627842076895,
-13.3214909282701));
#60998=CARTESIAN_POINT('Ctrl Pts',(-16.3053772882528,-18.1424373254742,
-13.3256662130195));
#60999=CARTESIAN_POINT('Ctrl Pts',(-16.2788072794351,-18.2221452083798,
-13.329844368466));
#61000=CARTESIAN_POINT('Ctrl Pts',(-16.2561931190383,-18.3030793228292,
-13.3340225239125));
#61001=CARTESIAN_POINT('Ctrl Pts',(-16.2376231931974,-18.3848114612778,
-13.338200679359));
#61002=CARTESIAN_POINT('Ctrl Pts',(-16.2190239659388,-18.4666725645667,
-13.3423854275016));
#61003=CARTESIAN_POINT('Ctrl Pts',(-16.2044817823337,-18.549333752171,-13.3465701756442));
#61004=CARTESIAN_POINT('Ctrl Pts',(-16.1940334157616,-18.6323599665996,
-13.3507549237868));
#61005=CARTESIAN_POINT('Ctrl Pts',(-16.1917823436453,-18.6502477383323,
-13.3516565163747));
#61006=CARTESIAN_POINT('Ctrl Pts',(-16.1897211040228,-18.6681524506455,
-13.3525581089627));
#61007=CARTESIAN_POINT('Ctrl Pts',(-16.1878497481281,-18.6860697555883,
-13.3534597015506));
#61008=CARTESIAN_POINT('Ctrl Pts',(-16.1791640730867,-18.7692307880738,
-13.3576443359436));
#61009=CARTESIAN_POINT('Ctrl Pts',(-16.1745407622114,-18.852972557727,-13.3618289703367));
#61010=CARTESIAN_POINT('Ctrl Pts',(-16.1740447460464,-18.9368640244713,
-13.3660136047297));
#61011=CARTESIAN_POINT('Ctrl Pts',(-16.173549435899,-19.0206360820962,-13.3701922828137));
#61012=CARTESIAN_POINT('Ctrl Pts',(-16.1771697541693,-19.1045569574875,
-13.3743709608976));
#61013=CARTESIAN_POINT('Ctrl Pts',(-16.1849189310736,-19.1881899744724,
-13.3785496389816));
#61014=CARTESIAN_POINT('Ctrl Pts',(-16.1928070064048,-19.2733220531809,
-13.382803216867));
#61015=CARTESIAN_POINT('Ctrl Pts',(-16.2049734659499,-19.3581553727241,
-13.3870567947524));
#61016=CARTESIAN_POINT('Ctrl Pts',(-16.2213767120001,-19.4422287349806,
-13.3913103726379));
#61017=CARTESIAN_POINT('Ctrl Pts',(-16.2374619491174,-19.5246721710542,
-13.3954814866158));
#61018=CARTESIAN_POINT('Ctrl Pts',(-16.2576210698179,-19.6063843810837,
-13.3996526005938));
#61019=CARTESIAN_POINT('Ctrl Pts',(-16.2817626998464,-19.686936884185,-13.4038237145717));
#61020=CARTESIAN_POINT('Ctrl Pts',(-16.3058962289179,-19.7674623571159,
-13.4079934288921));
#61021=CARTESIAN_POINT('Ctrl Pts',(-16.334009481308,-19.8468284556772,-13.4121631432125));
#61022=CARTESIAN_POINT('Ctrl Pts',(-16.3659607754928,-19.9246202913754,
-13.4163328575329));
#61023=CARTESIAN_POINT('Ctrl Pts',(-16.3979109327134,-20.0024093589062,
-13.4205024234769));
#61024=CARTESIAN_POINT('Ctrl Pts',(-16.4336986846161,-20.0786238497405,
-13.4246719894209));
#61025=CARTESIAN_POINT('Ctrl Pts',(-16.4731341172713,-20.1528686274167,
-13.428841555365));
#61026=CARTESIAN_POINT('Ctrl Pts',(-16.5139560510899,-20.2297237598851,
-13.4331577181039));
#61027=CARTESIAN_POINT('Ctrl Pts',(-16.5586866956795,-20.3044676260571,
-13.4374738808428));
#61028=CARTESIAN_POINT('Ctrl Pts',(-16.6070644247003,-20.3766912151497,
-13.4417900435817));
#61029=CARTESIAN_POINT('Ctrl Pts',(-16.6538662542869,-20.4465621284242,
-13.4459656077734));
#61030=CARTESIAN_POINT('Ctrl Pts',(-16.7040808906406,-20.514074089366,-13.4501411719651));
#61031=CARTESIAN_POINT('Ctrl Pts',(-16.75742932982,-20.5788891744013,-13.4543167361568));
#61032=CARTESIAN_POINT('Ctrl Pts',(-16.8134722718384,-20.6469779152985,
-13.4587031981693));
#61033=CARTESIAN_POINT('Ctrl Pts',(-16.8729735193545,-20.7120897510531,
-13.4630896601819));
#61034=CARTESIAN_POINT('Ctrl Pts',(-16.9355661330672,-20.7738769514621,
-13.4674761221944));
#61035=CARTESIAN_POINT('Ctrl Pts',(-16.9981587467798,-20.8356641518712,
-13.4718625842069));
#61036=CARTESIAN_POINT('Ctrl Pts',(-17.0638422427094,-20.8941263879947,
-13.4762490462195));
#61037=CARTESIAN_POINT('Ctrl Pts',(-17.1322119090441,-20.9489664272771,
-13.480635508232));
#61038=CARTESIAN_POINT('Ctrl Pts',(-17.1974357856827,-21.0012831950598,
-13.4848201426251));
#61039=CARTESIAN_POINT('Ctrl Pts',(-17.2653468510499,-21.0504984994761,
-13.4890047770181));
#61040=CARTESIAN_POINT('Ctrl Pts',(-17.3356178143268,-21.0963244303957,
-13.4931894114112));
#61041=CARTESIAN_POINT('Ctrl Pts',(-17.4057887555854,-21.1420851337748,
-13.4973680894951));
#61042=CARTESIAN_POINT('Ctrl Pts',(-17.4783125406379,-21.1844657972013,
-13.5015467675791));
#61043=CARTESIAN_POINT('Ctrl Pts',(-17.552829155194,-21.2232189316269,-13.505725445663));
#61044=CARTESIAN_POINT('Ctrl Pts',(-17.6286814265118,-21.2626666881356,
-13.5099790235484));
#61045=CARTESIAN_POINT('Ctrl Pts',(-17.7065982968803,-21.2983552879197,
-13.5142326014339));
#61046=CARTESIAN_POINT('Ctrl Pts',(-17.7861694556149,-21.3300700702735,
-13.5184861793193));
#61047=CARTESIAN_POINT('Ctrl Pts',(-17.864197972167,-21.361169999685,-13.5226572932973));
#61048=CARTESIAN_POINT('Ctrl Pts',(-17.9438167592515,-21.3884486389203,
-13.5268284072752));
#61049=CARTESIAN_POINT('Ctrl Pts',(-18.0246160731019,-21.4117508906917,
-13.5309995212532));
#61050=CARTESIAN_POINT('Ctrl Pts',(-18.1053882739622,-21.4350453231675,
-13.5351692355736));
#61051=CARTESIAN_POINT('Ctrl Pts',(-18.1873397732036,-21.4543658907802,
-13.5393389498939));
#61052=CARTESIAN_POINT('Ctrl Pts',(-18.2700450257389,-21.4696071539973,
-13.5435086642143));
#61053=CARTESIAN_POINT('Ctrl Pts',(-18.3527473352663,-21.4848478748648,
-13.5476782301583));
#61054=CARTESIAN_POINT('Ctrl Pts',(-18.4362028921898,-21.4960094974156,
-13.5518477961024));
#61055=CARTESIAN_POINT('Ctrl Pts',(-18.5199766524688,-21.5030378293376,
-13.5560173620464));
#61056=CARTESIAN_POINT('Ctrl Pts',(-18.6066957948131,-21.5103132687396,
-13.5603335247854));
#61057=CARTESIAN_POINT('Ctrl Pts',(-18.6937554073231,-21.5131593125471,
-13.5646496875243));
#61058=CARTESIAN_POINT('Ctrl Pts',(-18.780669963282,-21.5115745573293,-13.5689658502632));
#61059=CARTESIAN_POINT('Ctrl Pts',(-18.8647532867224,-21.5100414253459,
-13.5731414144549));
#61060=CARTESIAN_POINT('Ctrl Pts',(-18.9487003921373,-21.5043618068031,
-13.5773169786466));
#61061=CARTESIAN_POINT('Ctrl Pts',(-19.032076119737,-21.4945873882411,-13.5814925428382));
#61062=CARTESIAN_POINT('Ctrl Pts',(-19.1196629571309,-21.484319287034,-13.5858790048508));
#61063=CARTESIAN_POINT('Ctrl Pts',(-19.2066186035792,-21.4695319558998,
-13.5902654668633));
#61064=CARTESIAN_POINT('Ctrl Pts',(-19.2924520557266,-21.4503457129578,
-13.5946519288759));
#61065=CARTESIAN_POINT('Ctrl Pts',(-19.378285507874,-21.4311594700159,-13.5990383908884));
#61066=CARTESIAN_POINT('Ctrl Pts',(-19.4629962271651,-21.4075745441673,
-13.6034248529009));
#61067=CARTESIAN_POINT('Ctrl Pts',(-19.546115225231,-21.379770347654,-13.6078113149135));
#61068=CARTESIAN_POINT('Ctrl Pts',(-19.6254097949839,-21.353245463438,-13.6119959493065));
#61069=CARTESIAN_POINT('Ctrl Pts',(-19.7035510491552,-21.3227823154618,
-13.6161805836996));
#61070=CARTESIAN_POINT('Ctrl Pts',(-19.7801197445754,-21.2885002632162,
-13.6203652180926));
#61071=CARTESIAN_POINT('Ctrl Pts',(-19.856579453935,-21.2542670072287,-13.6245438961766));
#61072=CARTESIAN_POINT('Ctrl Pts',(-19.9314706343177,-21.2162258304373,
-13.6287225742605));
#61073=CARTESIAN_POINT('Ctrl Pts',(-20.0043903176929,-21.1745454867588,
-13.6329012523444));
#61074=CARTESIAN_POINT('Ctrl Pts',(-20.0786170339862,-21.1321180528751,
-13.6371548302299));
#61075=CARTESIAN_POINT('Ctrl Pts',(-20.1508004226815,-21.0859198576825,
-13.6414084081153));
#61076=CARTESIAN_POINT('Ctrl Pts',(-20.2205378947045,-21.0361797157653,
-13.6456619860007));
#61077=CARTESIAN_POINT('Ctrl Pts',(-20.2889233697509,-20.9874038835591,
-13.6498330999787));
#61078=CARTESIAN_POINT('Ctrl Pts',(-20.3549565277685,-20.935222493605,-13.6540042139566));
#61079=CARTESIAN_POINT('Ctrl Pts',(-20.418285169954,-20.8798961243472,-13.6581753279346));
#61080=CARTESIAN_POINT('Ctrl Pts',(-20.4815925616021,-20.8245883203869,
-13.662345042255));
#61081=CARTESIAN_POINT('Ctrl Pts',(-20.5421968936245,-20.7661379354361,
-13.6665147565753));
#61082=CARTESIAN_POINT('Ctrl Pts',(-20.599779168576,-20.7048457131499,-13.6706844708957));
#61083=CARTESIAN_POINT('Ctrl Pts',(-20.657359394503,-20.643555671904,-13.6748540368397));
#61084=CARTESIAN_POINT('Ctrl Pts',(-20.711917462806,-20.5794243302495,-13.6790236027838));
#61085=CARTESIAN_POINT('Ctrl Pts',(-20.7631723252387,-20.5127881581065,
-13.6831931687278));
#61086=CARTESIAN_POINT('Ctrl Pts',(-20.816229245405,-20.4438091403553,-13.6875093314667));
#61087=CARTESIAN_POINT('Ctrl Pts',(-20.8657460348865,-20.3721462932503,
-13.6918254942057));
#61088=CARTESIAN_POINT('Ctrl Pts',(-20.9114587072169,-20.2982071082733,
-13.6961416569446));
#61089=CARTESIAN_POINT('Ctrl Pts',(-20.9556822940541,-20.22667648447,-13.7003172211363));
#61090=CARTESIAN_POINT('Ctrl Pts',(-20.9963456096571,-20.1530159839388,
-13.7044927853279));
#61091=CARTESIAN_POINT('Ctrl Pts',(-21.0332565704857,-20.0776194841413,
-13.7086683495196));
#61092=CARTESIAN_POINT('Ctrl Pts',(-21.0720318161984,-19.998414886377,-13.7130548115322));
#61093=CARTESIAN_POINT('Ctrl Pts',(-21.1066654530387,-19.9172948468642,
-13.7174412735447));
#61094=CARTESIAN_POINT('Ctrl Pts',(-21.1369928787005,-19.8347373476378,
-13.7218277355573));
#61095=CARTESIAN_POINT('Ctrl Pts',(-21.1673203043624,-19.7521798484114,
-13.7262141975698));
#61096=CARTESIAN_POINT('Ctrl Pts',(-21.1933414198056,-19.6681854662111,
-13.7306006595824));
#61097=CARTESIAN_POINT('Ctrl Pts',(-21.214953227824,-19.5832456584798,-13.7349871215949));
#61098=CARTESIAN_POINT('Ctrl Pts',(-21.2416966549182,-19.4781373050501,
-13.740415127754));
#61099=CARTESIAN_POINT('Ctrl Pts',(-21.261771847948,-19.3712684537292,-13.7458431339132));
#61100=CARTESIAN_POINT('Ctrl Pts',(-21.2749934581328,-19.2633715557439,
-13.7512711400723));
#61101=CARTESIAN_POINT('Ctrl Pts',(-21.2875287526693,-19.1610754377283,
-13.7564173858775));
#61102=CARTESIAN_POINT('Ctrl Pts',(-21.2939037306885,-19.05785506064,-13.7615636316826));
#61103=CARTESIAN_POINT('Ctrl Pts',(-21.2939989173812,-18.9543543592142,
-13.7667098774877));
#61104=CARTESIAN_POINT('Origin',(-18.734,-18.952,1.76670989022851));
#61105=CARTESIAN_POINT('',(-17.1725834092545,-16.9193794902115,-12.4500366838548));
#61106=CARTESIAN_POINT('',(-17.1744641548914,-16.9218650419685,-12.516719348784));
#61107=CARTESIAN_POINT('',(-17.1744641548914,-16.9218650419685,1.76670989022851));
#61108=CARTESIAN_POINT('',(-21.293999998394,-18.9520906788001,-13.0332901097364));
#61109=CARTESIAN_POINT('Ctrl Pts',(-17.1744641548914,-16.9218650419685,
-12.516719348784));
#61110=CARTESIAN_POINT('Ctrl Pts',(-17.1077873931624,-16.9730856761145,
-12.5208888646352));
#61111=CARTESIAN_POINT('Ctrl Pts',(-17.0436201053814,-17.0276073338008,
-12.5250583804865));
#61112=CARTESIAN_POINT('Ctrl Pts',(-16.9822975341889,-17.0851474425463,
-12.5292278963377));
#61113=CARTESIAN_POINT('Ctrl Pts',(-16.9209704681146,-17.1426917689231,
-12.5333977178102));
#61114=CARTESIAN_POINT('Ctrl Pts',(-16.8624888672419,-17.2032546699353,
-12.5375675392827));
#61115=CARTESIAN_POINT('Ctrl Pts',(-16.8071519907267,-17.2665158709856,
-12.5417373607552));
#61116=CARTESIAN_POINT('Ctrl Pts',(-16.7517572859962,-17.3298431813393,
-12.5459115397801));
#61117=CARTESIAN_POINT('Ctrl Pts',(-16.6995141714666,-17.3958740754972,
-12.5500857188049));
#61118=CARTESIAN_POINT('Ctrl Pts',(-16.6506820340232,-17.4642546411976,
-12.5542598978297));
#61119=CARTESIAN_POINT('Ctrl Pts',(-16.6018236009596,-17.5326720291522,
-12.5584363246084));
#61120=CARTESIAN_POINT('Ctrl Pts',(-16.5563800512887,-17.60344122091,-12.5626127513871));
#61121=CARTESIAN_POINT('Ctrl Pts',(-16.5145664411709,-17.6761807816375,
-12.5667891781657));
#61122=CARTESIAN_POINT('Ctrl Pts',(-16.4726799830268,-17.7490470698447,
-12.5709728811506));
#61123=CARTESIAN_POINT('Ctrl Pts',(-16.4344363059152,-17.8238901736935,
-12.5751565841354));
#61124=CARTESIAN_POINT('Ctrl Pts',(-16.4000035693677,-17.9003058135581,
-12.5793402871203));
#61125=CARTESIAN_POINT('Ctrl Pts',(-16.3735296901039,-17.9590585769595,
-12.5825569599381));
#61126=CARTESIAN_POINT('Ctrl Pts',(-16.3493076566629,-18.0187404532435,
-12.585773632756));
#61127=CARTESIAN_POINT('Ctrl Pts',(-16.3273937923111,-18.0791617783844,
-12.5889903055738));
#61128=CARTESIAN_POINT('Ctrl Pts',(-16.2988856052357,-18.1577650960284,
-12.5931749399669));
#61129=CARTESIAN_POINT('Ctrl Pts',(-16.2741793660911,-18.2379128391993,
-12.5973595743599));
#61130=CARTESIAN_POINT('Ctrl Pts',(-16.2534421603043,-18.3192023989267,
-12.601544208753));
#61131=CARTESIAN_POINT('Ctrl Pts',(-16.2327344713632,-18.4003762530275,
-12.6057228868369));
#61132=CARTESIAN_POINT('Ctrl Pts',(-16.2159847069801,-18.482688253513,-12.6099015649209));
#61133=CARTESIAN_POINT('Ctrl Pts',(-16.2033111427937,-18.5657178388638,
-12.6140802430048));
#61134=CARTESIAN_POINT('Ctrl Pts',(-16.1904104140776,-18.6502356698597,
-12.6183338208902));
#61135=CARTESIAN_POINT('Ctrl Pts',(-16.1817336190671,-18.7354966109226,
-12.6225873987757));
#61136=CARTESIAN_POINT('Ctrl Pts',(-16.177351748603,-18.8210430657489,-12.6268409766611));
#61137=CARTESIAN_POINT('Ctrl Pts',(-16.1730548292482,-18.9049310356181,
-12.6310120906391));
#61138=CARTESIAN_POINT('Ctrl Pts',(-16.1728878141637,-18.9890930669701,
-12.635183204617));
#61139=CARTESIAN_POINT('Ctrl Pts',(-16.1768654907269,-19.0730912940078,
-12.639354318595));
#61140=CARTESIAN_POINT('Ctrl Pts',(-16.1808418325422,-19.1570613346291,
-12.6435240329153));
#61141=CARTESIAN_POINT('Ctrl Pts',(-16.1889600821296,-19.2408672209642,
-12.6476937472357));
#61142=CARTESIAN_POINT('Ctrl Pts',(-16.2011829261396,-19.3240721305891,
-12.6518634615561));
#61143=CARTESIAN_POINT('Ctrl Pts',(-16.2134053352083,-19.4072740794261,
-12.6560330275001));
#61144=CARTESIAN_POINT('Ctrl Pts',(-16.229731980592,-19.4898746390482,-12.6602025934442));
#61145=CARTESIAN_POINT('Ctrl Pts',(-16.250073974422,-19.5714445087789,-12.6643721593882));
#61146=CARTESIAN_POINT('Ctrl Pts',(-16.2711311676606,-19.6558822745023,
-12.6686883221271));
#61147=CARTESIAN_POINT('Ctrl Pts',(-16.2964911945897,-19.7392150119464,
-12.6730044848661));
#61148=CARTESIAN_POINT('Ctrl Pts',(-16.3259989267241,-19.8209826414273,
-12.677320647605));
#61149=CARTESIAN_POINT('Ctrl Pts',(-16.3545454475878,-19.9000866989782,
-12.6814962117967));
#61150=CARTESIAN_POINT('Ctrl Pts',(-16.3869733753121,-19.9777256330116,
-12.6856717759884));
#61151=CARTESIAN_POINT('Ctrl Pts',(-16.4230935537342,-20.0535041518792,
-12.68984734018));
#61152=CARTESIAN_POINT('Ctrl Pts',(-16.4610380765009,-20.1331100635887,
-12.6942338021926));
#61153=CARTESIAN_POINT('Ctrl Pts',(-16.5030573653642,-20.2106621684909,
-12.6986202642051));
#61154=CARTESIAN_POINT('Ctrl Pts',(-16.5488792984353,-20.2857344261859,
-12.7030067262177));
#61155=CARTESIAN_POINT('Ctrl Pts',(-16.5947012315064,-20.3608066838809,
-12.7073931882302));
#61156=CARTESIAN_POINT('Ctrl Pts',(-16.6443254185492,-20.4333986583029,
-12.7117796502428));
#61157=CARTESIAN_POINT('Ctrl Pts',(-16.6974308899397,-20.5031241923032,
-12.7161661122553));
#61158=CARTESIAN_POINT('Ctrl Pts',(-16.7480928998703,-20.5696415511261,
-12.7203507466484));
#61159=CARTESIAN_POINT('Ctrl Pts',(-16.8021114495637,-20.6337980416559,
-12.7245353810414));
#61160=CARTESIAN_POINT('Ctrl Pts',(-16.8592384487626,-20.6952352468906,
-12.7287200154345));
#61161=CARTESIAN_POINT('Ctrl Pts',(-16.916284134749,-20.7565850038681,-12.7328986935184));
#61162=CARTESIAN_POINT('Ctrl Pts',(-16.9764291712246,-20.8152228296987,
-12.7370773716024));
#61163=CARTESIAN_POINT('Ctrl Pts',(-17.0393839528669,-20.8708216313141,
-12.7412560496863));
#61164=CARTESIAN_POINT('Ctrl Pts',(-17.1034671537253,-20.9274170014903,
-12.7455096275717));
#61165=CARTESIAN_POINT('Ctrl Pts',(-17.1704615277519,-20.9808629432572,
-12.7497632054572));
#61166=CARTESIAN_POINT('Ctrl Pts',(-17.2400207348673,-21.0308520763521,
-12.7540167833426));
#61167=CARTESIAN_POINT('Ctrl Pts',(-17.308231401019,-21.0798720725562,-12.7581878973205));
#61168=CARTESIAN_POINT('Ctrl Pts',(-17.3789079483581,-21.1255678171231,
-12.7623590112985));
#61169=CARTESIAN_POINT('Ctrl Pts',(-17.4516902051702,-21.1676898677575,
-12.7665301252764));
#61170=CARTESIAN_POINT('Ctrl Pts',(-17.524448039193,-21.2097977839311,-12.7706998395968));
#61171=CARTESIAN_POINT('Ctrl Pts',(-17.5993097815587,-21.2483341575378,
-12.7748695539172));
#61172=CARTESIAN_POINT('Ctrl Pts',(-17.6758879367288,-21.2830939195064,
-12.7790392682375));
#61173=CARTESIAN_POINT('Ctrl Pts',(-17.7524633669194,-21.3178524445735,
-12.7832088341816));
#61174=CARTESIAN_POINT('Ctrl Pts',(-17.8307546692264,-21.3488344358334,
-12.7873784001256));
#61175=CARTESIAN_POINT('Ctrl Pts',(-17.910352756402,-21.375882261603,-12.7915479660697));
#61176=CARTESIAN_POINT('Ctrl Pts',(-17.9927494141279,-21.4038810555595,
-12.7958641288086));
#61177=CARTESIAN_POINT('Ctrl Pts',(-18.0765459602124,-21.4276637164715,
-12.8001802915475));
#61178=CARTESIAN_POINT('Ctrl Pts',(-18.1612715723437,-21.4471116504386,
-12.8044964542864));
#61179=CARTESIAN_POINT('Ctrl Pts',(-18.2432372565715,-21.4659260700023,
-12.8086720184781));
#61180=CARTESIAN_POINT('Ctrl Pts',(-18.3260719356987,-21.4806837970704,
-12.8128475826698));
#61181=CARTESIAN_POINT('Ctrl Pts',(-18.4093408453622,-21.4913299181693,
-12.8170231468614));
#61182=CARTESIAN_POINT('Ctrl Pts',(-18.4968154696998,-21.5025137495362,
-12.821409608874));
#61183=CARTESIAN_POINT('Ctrl Pts',(-18.5847687611385,-21.5091596607904,
-12.8257960708865));
#61184=CARTESIAN_POINT('Ctrl Pts',(-18.6726951927072,-21.5112658557881,
-12.8301825328991));
#61185=CARTESIAN_POINT('Ctrl Pts',(-18.7606216242758,-21.5133720507858,
-12.8345689949116));
#61186=CARTESIAN_POINT('Ctrl Pts',(-18.8485206180845,-21.5109386216197,
-12.8389554569241));
#61187=CARTESIAN_POINT('Ctrl Pts',(-18.9358937423124,-21.5040264334084,
-12.8433419189367));
#61188=CARTESIAN_POINT('Ctrl Pts',(-19.0192466995766,-21.497432285223,-12.8475265533297));
#61189=CARTESIAN_POINT('Ctrl Pts',(-19.1024313715337,-21.4867379250515,
-12.8517111877228));
#61190=CARTESIAN_POINT('Ctrl Pts',(-19.1850120996547,-21.4719579532137,
-12.8558958221158));
#61191=CARTESIAN_POINT('Ctrl Pts',(-19.2674752843307,-21.4571990188365,
-12.8600745001998));
#61192=CARTESIAN_POINT('Ctrl Pts',(-19.3493357837206,-21.4383661042867,
-12.8642531782837));
#61193=CARTESIAN_POINT('Ctrl Pts',(-19.4301618064492,-21.4155256725355,
-12.8684318563676));
#61194=CARTESIAN_POINT('Ctrl Pts',(-19.5124365775465,-21.3922758424603,
-12.8726854342531));
#61195=CARTESIAN_POINT('Ctrl Pts',(-19.5936389405807,-21.3648734505894,
-12.8769390121385));
#61196=CARTESIAN_POINT('Ctrl Pts',(-19.6733229700786,-21.333443335014,-12.881192590024));
#61197=CARTESIAN_POINT('Ctrl Pts',(-19.7514621691741,-21.3026225535599,
-12.8853637040019));
#61198=CARTESIAN_POINT('Ctrl Pts',(-19.8281409334346,-21.2679290018995,
-12.8895348179799));
#61199=CARTESIAN_POINT('Ctrl Pts',(-19.9029545672469,-21.229530509063,-12.8937059319578));
#61200=CARTESIAN_POINT('Ctrl Pts',(-19.9777430966217,-21.1911449012116,
-12.8978756462782));
#61201=CARTESIAN_POINT('Ctrl Pts',(-20.0506673295889,-21.1490570311429,
-12.9020453605985));
#61202=CARTESIAN_POINT('Ctrl Pts',(-20.1213450915269,-21.1034817212833,
-12.9062150749189));
#61203=CARTESIAN_POINT('Ctrl Pts',(-20.1920203384467,-21.0579080331889,
-12.9103846408629));
#61204=CARTESIAN_POINT('Ctrl Pts',(-20.2604488871165,-21.008847402065,-12.914554206807));
#61205=CARTESIAN_POINT('Ctrl Pts',(-20.3262767630685,-20.9565584825073,
-12.918723772751));
#61206=CARTESIAN_POINT('Ctrl Pts',(-20.3944190659317,-20.9024311490432,
-12.9230399354899));
#61207=CARTESIAN_POINT('Ctrl Pts',(-20.4597740011395,-20.8448446181548,
-12.9273560982289));
#61208=CARTESIAN_POINT('Ctrl Pts',(-20.521987002802,-20.7841305842682,-12.9316722609678));
#61209=CARTESIAN_POINT('Ctrl Pts',(-20.582173422479,-20.7253943036496,-12.9358478251595));
#61210=CARTESIAN_POINT('Ctrl Pts',(-20.63941917621,-20.6637315251353,-12.9400233893512));
#61211=CARTESIAN_POINT('Ctrl Pts',(-20.6934427607502,-20.5994780931301,
-12.9441989535428));
#61212=CARTESIAN_POINT('Ctrl Pts',(-20.7501949481167,-20.5319793730223,
-12.9485854155554));
#61213=CARTESIAN_POINT('Ctrl Pts',(-20.803390556233,-20.4616218795445,-12.9529718775679));
#61214=CARTESIAN_POINT('Ctrl Pts',(-20.852754442665,-20.3888297086597,-12.9573583395805));
#61215=CARTESIAN_POINT('Ctrl Pts',(-20.9021183290971,-20.316037537775,-12.961744801593));
#61216=CARTESIAN_POINT('Ctrl Pts',(-20.9476502584794,-20.240811225245,-12.9661312636056));
#61217=CARTESIAN_POINT('Ctrl Pts',(-20.9891316170535,-20.1636028184871,
-12.9705177256181));
#61218=CARTESIAN_POINT('Ctrl Pts',(-21.0308618762442,-20.0859311380874,
-12.9749305077209));
#61219=CARTESIAN_POINT('Ctrl Pts',(-21.0686351706121,-20.0059905501583,
-12.9793432898236));
#61220=CARTESIAN_POINT('Ctrl Pts',(-21.1022126120118,-19.9241980375974,
-12.9837560719264));
#61221=CARTESIAN_POINT('Ctrl Pts',(-21.1356929152447,-19.8426421474353,
-12.9881560880307));
#61222=CARTESIAN_POINT('Ctrl Pts',(-21.1650014030469,-19.759245362016,-12.9925561041351));
#61223=CARTESIAN_POINT('Ctrl Pts',(-21.1899457627449,-19.6744475139796,
-12.9969561202394));
#61224=CARTESIAN_POINT('Ctrl Pts',(-21.2148467487816,-19.5897971138308,
-13.0013484855236));
#61225=CARTESIAN_POINT('Ctrl Pts',(-21.235398596884,-19.5037508664335,-13.0057408508078));
#61226=CARTESIAN_POINT('Ctrl Pts',(-21.2514572537729,-19.4167676574658,
-13.0101332160921));
#61227=CARTESIAN_POINT('Ctrl Pts',(-21.2674789983323,-19.3299843875645,
-13.0145154851126));
#61228=CARTESIAN_POINT('Ctrl Pts',(-21.2790280568698,-19.2422688247272,
-13.0188977541331));
#61229=CARTESIAN_POINT('Ctrl Pts',(-21.2860106924303,-19.1540926166924,
-13.0232800231537));
#61230=CARTESIAN_POINT('Ctrl Pts',(-21.2913273283411,-19.0869545296399,
-13.0266167186812));
#61231=CARTESIAN_POINT('Ctrl Pts',(-21.2939976088987,-19.0195497546626,
-13.0299534142088));
#61232=CARTESIAN_POINT('Ctrl Pts',(-21.293999998394,-18.9520906788001,-13.0332901097364));
#61233=CARTESIAN_POINT('Ctrl Pts',(-21.293999998394,-18.9520906780896,-13.0332901097715));
#61234=CARTESIAN_POINT('Ctrl Pts',(-21.2940031178915,-18.8640218456489,
-13.0376462156856));
#61235=CARTESIAN_POINT('Ctrl Pts',(-21.2894573285641,-18.7760356076548,
-13.0420023215996));
#61236=CARTESIAN_POINT('Ctrl Pts',(-21.2804139262416,-18.6886065372051,
-13.0463584275137));
#61237=CARTESIAN_POINT('Ctrl Pts',(-21.2713470661108,-18.600950683262,-13.0507258327921));
#61238=CARTESIAN_POINT('Ctrl Pts',(-21.2577593163574,-18.5138552818864,
-13.0550932380704));
#61239=CARTESIAN_POINT('Ctrl Pts',(-21.2397536148681,-18.4277874271106,
-13.0594606433487));
#61240=CARTESIAN_POINT('Ctrl Pts',(-21.2217244341812,-18.3416073409855,
-13.0638337436661));
#61241=CARTESIAN_POINT('Ctrl Pts',(-21.1992659159007,-18.25645785704,-13.0682068439834));
#61242=CARTESIAN_POINT('Ctrl Pts',(-21.172530963322,-18.1727909517209,-13.0725799443007));
#61243=CARTESIAN_POINT('Ctrl Pts',(-21.1457232584229,-18.0888963683656,
-13.0769649448896));
#61244=CARTESIAN_POINT('Ctrl Pts',(-21.114615990053,-18.0064928038113,-13.0813499454785));
#61245=CARTESIAN_POINT('Ctrl Pts',(-21.0794107185113,-17.9260133716796,
-13.0857349460673));
#61246=CARTESIAN_POINT('Ctrl Pts',(-21.0474072811094,-17.8528533488881,
-13.0897211414781));
#61247=CARTESIAN_POINT('Ctrl Pts',(-21.0120180507083,-17.7812832866316,
-13.0937073368888));
#61248=CARTESIAN_POINT('Ctrl Pts',(-20.9734262024016,-17.7116088181557,
-13.0976935322996));
#61249=CARTESIAN_POINT('Ctrl Pts',(-20.9329131921061,-17.6384658467109,
-13.1018781666926));
#61250=CARTESIAN_POINT('Ctrl Pts',(-20.8887375841054,-17.5671736686977,
-13.1060628010857));
#61251=CARTESIAN_POINT('Ctrl Pts',(-20.8410930440999,-17.4981228031551,
-13.1102474354787));
#61252=CARTESIAN_POINT('Ctrl Pts',(-20.7935163201999,-17.4291702229727,
-13.1144261135626));
#61253=CARTESIAN_POINT('Ctrl Pts',(-20.7424807309408,-17.3624529938651,
-13.1186047916466));
#61254=CARTESIAN_POINT('Ctrl Pts',(-20.6882255495785,-17.2983366420657,
-13.1227834697305));
#61255=CARTESIAN_POINT('Ctrl Pts',(-20.6329978830829,-17.23307105074,-13.127037047616));
#61256=CARTESIAN_POINT('Ctrl Pts',(-20.5744343004281,-17.1705009170561,
-13.1312906255014));
#61257=CARTESIAN_POINT('Ctrl Pts',(-20.5128330635401,-17.1109804639666,
-13.1355442033868));
#61258=CARTESIAN_POINT('Ctrl Pts',(-20.4524260868341,-17.0526139310049,
-13.1397153173648));
#61259=CARTESIAN_POINT('Ctrl Pts',(-20.3890985326089,-16.9971802202218,
-13.1438864313427));
#61260=CARTESIAN_POINT('Ctrl Pts',(-20.323170725482,-16.9449782250132,-13.1480575453207));
#61261=CARTESIAN_POINT('Ctrl Pts',(-20.2572650410674,-16.8927937466883,
-13.1522272596411));
#61262=CARTESIAN_POINT('Ctrl Pts',(-20.1887611969918,-16.8438391155729,
-13.1563969739614));
#61263=CARTESIAN_POINT('Ctrl Pts',(-20.1180129698811,-16.7983732683678,
-13.1605666882818));
#61264=CARTESIAN_POINT('Ctrl Pts',(-20.0472672602961,-16.7529090390327,
-13.1647362542259));
#61265=CARTESIAN_POINT('Ctrl Pts',(-19.9742777139359,-16.7109335947646,
-13.1689058201699));
#61266=CARTESIAN_POINT('Ctrl Pts',(-19.8994263305447,-16.672662054878,-13.1730753861139));
#61267=CARTESIAN_POINT('Ctrl Pts',(-19.8219432648525,-16.6330449348619,
-13.1773915488529));
#61268=CARTESIAN_POINT('Ctrl Pts',(-19.7424654713775,-16.5973972639687,
-13.1817077115918));
#61269=CARTESIAN_POINT('Ctrl Pts',(-19.6614416802126,-16.5659044592045,
-13.1860238743307));
#61270=CARTESIAN_POINT('Ctrl Pts',(-19.5830572305228,-16.535437529243,-13.1901994385224));
#61271=CARTESIAN_POINT('Ctrl Pts',(-19.5032264199663,-16.5088590368059,
-13.1943750027141));
#61272=CARTESIAN_POINT('Ctrl Pts',(-19.4223715061057,-16.4862861744351,
-13.1985505669057));
#61273=CARTESIAN_POINT('Ctrl Pts',(-19.3374328027602,-16.4625732104478,
-13.2029370289183));
#61274=CARTESIAN_POINT('Ctrl Pts',(-19.2513643920954,-16.4432812873466,
-13.2073234909308));
#61275=CARTESIAN_POINT('Ctrl Pts',(-19.1646662302708,-16.4284852688949,
-13.2117099529434));
#61276=CARTESIAN_POINT('Ctrl Pts',(-19.0779680684462,-16.4136892504433,
-13.2160964149559));
#61277=CARTESIAN_POINT('Ctrl Pts',(-18.9906407405946,-16.4033891290646,
-13.2204828769685));
#61278=CARTESIAN_POINT('Ctrl Pts',(-18.9031862415112,-16.3975967398073,
-13.224869338981));
#61279=CARTESIAN_POINT('Ctrl Pts',(-18.8197759389863,-16.3920722105337,
-13.2290529559168));
#61280=CARTESIAN_POINT('Ctrl Pts',(-18.7359395737696,-16.3906271591048,
-13.2332365728527));
#61281=CARTESIAN_POINT('Ctrl Pts',(-18.6521100212328,-16.3933100947208,
-13.2374201897885));
#61282=CARTESIAN_POINT('Ctrl Pts',(-18.5683906915468,-16.395989502693,-13.2415983059174));
#61283=CARTESIAN_POINT('Ctrl Pts',(-18.4846786121397,-16.4027861079029,
-13.2457764220463));
#61284=CARTESIAN_POINT('Ctrl Pts',(-18.401410469972,-16.4136965893503,-13.2499545381752));
#61285=CARTESIAN_POINT('Ctrl Pts',(-18.3182268241528,-16.4245959993866,
-13.2541284145607));
#61286=CARTESIAN_POINT('Ctrl Pts',(-18.2354866744767,-16.4396009359398,
-13.2583022909461));
#61287=CARTESIAN_POINT('Ctrl Pts',(-18.1536240274504,-16.4586561146751,
-13.2624761673316));
#61288=CARTESIAN_POINT('Ctrl Pts',(-18.0718198886652,-16.4776976744397,
-13.2666470605963));
#61289=CARTESIAN_POINT('Ctrl Pts',(-17.9908924531682,-16.5007836209311,
-13.2708179538609));
#61290=CARTESIAN_POINT('Ctrl Pts',(-17.9112665890683,-16.5278074056427,
-13.2749888471256));
#61291=CARTESIAN_POINT('Ctrl Pts',(-17.8316596834658,-16.554824756134,-13.2791587473226));
#61292=CARTESIAN_POINT('Ctrl Pts',(-17.7533541711449,-16.5857779414179,
-13.2833286475196));
#61293=CARTESIAN_POINT('Ctrl Pts',(-17.6767596812526,-16.6205105815349,
-13.2874985477166));
#61294=CARTESIAN_POINT('Ctrl Pts',(-17.6001752728535,-16.6552386500844,
-13.2916678990645));
#61295=CARTESIAN_POINT('Ctrl Pts',(-17.525301855604,-16.6937449890596,-13.2958372504123));
#61296=CARTESIAN_POINT('Ctrl Pts',(-17.4525274999375,-16.7358257668713,
-13.3000066017602));
#61297=CARTESIAN_POINT('Ctrl Pts',(-17.3797189214012,-16.7779263335904,
-13.3041779137873));
#61298=CARTESIAN_POINT('Ctrl Pts',(-17.3090117698551,-16.82360445842,-13.3083492258144));
#61299=CARTESIAN_POINT('Ctrl Pts',(-17.240767157218,-16.8726117059969,-13.3125205378415));
#61300=CARTESIAN_POINT('Ctrl Pts',(-17.2183978343134,-16.8886753761292,
-13.3138878168408));
#61301=CARTESIAN_POINT('Ctrl Pts',(-17.1962928438732,-16.9050963917938,
-13.31525509584));
#61302=CARTESIAN_POINT('Ctrl Pts',(-17.1744641548914,-16.9218650419685,
-13.3166223748392));
#61303=CARTESIAN_POINT('',(-21.2943301210028,-18.9513574887884,-12.9667098341108));
#61304=CARTESIAN_POINT('Ctrl Pts',(-21.2939999191096,-18.9513564484225,
-12.9667098902285));
#61305=CARTESIAN_POINT('Ctrl Pts',(-21.2939911726516,-18.9165636940744,
-12.9684506873211));
#61306=CARTESIAN_POINT('Ctrl Pts',(-21.2932731600888,-18.881780730387,-12.9701914844137));
#61307=CARTESIAN_POINT('Ctrl Pts',(-21.2918468828523,-18.8470270326106,
-12.9719322815063));
#61308=CARTESIAN_POINT('Ctrl Pts',(-21.2884183105029,-18.7634839708603,
-12.9761169158993));
#61309=CARTESIAN_POINT('Ctrl Pts',(-21.2808860937369,-18.6799535889704,
-12.9803015502924));
#61310=CARTESIAN_POINT('Ctrl Pts',(-21.2692483017375,-18.5968717857769,
-12.9844861846854));
#61311=CARTESIAN_POINT('Ctrl Pts',(-21.2576270746945,-18.5139082392468,
-12.9886648627694));
#61312=CARTESIAN_POINT('Ctrl Pts',(-21.2419119432712,-18.4313924548469,
-12.9928435408533));
#61313=CARTESIAN_POINT('Ctrl Pts',(-21.2221529486457,-18.3497584337279,
-12.9970222189372));
#61314=CARTESIAN_POINT('Ctrl Pts',(-21.2020397882419,-18.2666611814494,
-13.0012757968227));
#61315=CARTESIAN_POINT('Ctrl Pts',(-21.1777363859676,-18.1844780963255,
-13.0055293747081));
#61316=CARTESIAN_POINT('Ctrl Pts',(-21.1493505801536,-18.1036595170853,
-13.0097829525935));
#61317=CARTESIAN_POINT('Ctrl Pts',(-21.1215150885756,-18.0244077637083,
-13.0139540665715));
#61318=CARTESIAN_POINT('Ctrl Pts',(-21.0897542310845,-17.9464685351597,
-13.0181251805494));
#61319=CARTESIAN_POINT('Ctrl Pts',(-21.0542203695086,-17.8702526002261,
-13.0222962945274));
#61320=CARTESIAN_POINT('Ctrl Pts',(-21.0186984316631,-17.7940622402855,
-13.0264660088478));
#61321=CARTESIAN_POINT('Ctrl Pts',(-20.9794061983924,-17.7195944421082,
-13.0306357231681));
#61322=CARTESIAN_POINT('Ctrl Pts',(-20.9365438451406,-17.6472392517272,
-13.0348054374885));
#61323=CARTESIAN_POINT('Ctrl Pts',(-20.8936830171152,-17.5748866360543,
-13.0389750034325));
#61324=CARTESIAN_POINT('Ctrl Pts',(-20.8472525568965,-17.5046468740728,
-13.0431445693766));
#61325=CARTESIAN_POINT('Ctrl Pts',(-20.7974975099507,-17.4368834941077,
-13.0473141353206));
#61326=CARTESIAN_POINT('Ctrl Pts',(-20.7459931369336,-17.366737637298,-13.0516302980595));
#61327=CARTESIAN_POINT('Ctrl Pts',(-20.6909263546122,-17.2992459668448,
-13.0559464607985));
#61328=CARTESIAN_POINT('Ctrl Pts',(-20.6326151733211,-17.234775371818,-13.0602626235374));
#61329=CARTESIAN_POINT('Ctrl Pts',(-20.5762034726275,-17.1724048996433,
-13.0644381877291));
#61330=CARTESIAN_POINT('Ctrl Pts',(-20.5167558657732,-17.1128620023875,
-13.0686137519208));
#61331=CARTESIAN_POINT('Ctrl Pts',(-20.4545972806997,-17.0564407163983,
-13.0727893161124));
#61332=CARTESIAN_POINT('Ctrl Pts',(-20.3892992132619,-16.9971697253824,
-13.077175778125));
#61333=CARTESIAN_POINT('Ctrl Pts',(-20.3210095593889,-16.9413443477726,
-13.0815622401375));
#61334=CARTESIAN_POINT('Ctrl Pts',(-20.2501416763133,-16.889255610274,-13.0859487021501));
#61335=CARTESIAN_POINT('Ctrl Pts',(-20.1792737932376,-16.8371668727754,
-13.0903351641627));
#61336=CARTESIAN_POINT('Ctrl Pts',(-20.1058282074104,-16.7888150309008,
-13.0947216261752));
#61337=CARTESIAN_POINT('Ctrl Pts',(-20.0302483510417,-16.7444356832877,
-13.0991080881878));
#61338=CARTESIAN_POINT('Ctrl Pts',(-19.958146035901,-16.7020982952443,-13.1032927225808));
#61339=CARTESIAN_POINT('Ctrl Pts',(-19.8838331576254,-16.6632182861073,
-13.1074773569739));
#61340=CARTESIAN_POINT('Ctrl Pts',(-19.8076751930389,-16.6280332231607,
-13.1116619913669));
#61341=CARTESIAN_POINT('Ctrl Pts',(-19.7316256298885,-16.5928982417961,
-13.1158406694508));
#61342=CARTESIAN_POINT('Ctrl Pts',(-19.6537366110356,-16.5614479512896,
-13.1200193475348));
#61343=CARTESIAN_POINT('Ctrl Pts',(-19.5744001491065,-16.533875191521,-13.1241980256187));
#61344=CARTESIAN_POINT('Ctrl Pts',(-19.4936416381154,-16.5058082098496,
-13.1284516035042));
#61345=CARTESIAN_POINT('Ctrl Pts',(-19.4113836985809,-16.4817593798136,
-13.1327051813896));
#61346=CARTESIAN_POINT('Ctrl Pts',(-19.3280633649497,-16.461881786255,-13.136958759275));
#61347=CARTESIAN_POINT('Ctrl Pts',(-19.2463583585721,-16.4423895586354,
-13.141129873253));
#61348=CARTESIAN_POINT('Ctrl Pts',(-19.1636322517454,-16.4269083873419,
-13.1453009872309));
#61349=CARTESIAN_POINT('Ctrl Pts',(-19.0803129065813,-16.4155325015417,
-13.1494721012089));
#61350=CARTESIAN_POINT('Ctrl Pts',(-18.9970215200281,-16.4041604330299,
-13.1536418155293));
#61351=CARTESIAN_POINT('Ctrl Pts',(-18.9131377459122,-16.39689097632,-13.1578115298496));
#61352=CARTESIAN_POINT('Ctrl Pts',(-18.8290979023925,-16.3937669400618,
-13.16198124417));
#61353=CARTESIAN_POINT('Ctrl Pts',(-18.745061049371,-16.3906430149703,-13.1661508101141));
#61354=CARTESIAN_POINT('Ctrl Pts',(-18.6608685977346,-16.3916642332765,
-13.1703203760581));
#61355=CARTESIAN_POINT('Ctrl Pts',(-18.5769588557386,-16.3968213215102,
-13.1744899420021));
#61356=CARTESIAN_POINT('Ctrl Pts',(-18.4900989507279,-16.4021597266042,
-13.1788061047411));
#61357=CARTESIAN_POINT('Ctrl Pts',(-18.4035425318191,-16.4119302148937,
-13.18312226748));
#61358=CARTESIAN_POINT('Ctrl Pts',(-18.3177702276209,-16.4260639801085,
-13.1874384302189));
#61359=CARTESIAN_POINT('Ctrl Pts',(-18.2347919472102,-16.4397373394081,
-13.1916139944106));
#61360=CARTESIAN_POINT('Ctrl Pts',(-18.1525479314086,-16.4574939280207,
-13.1957895586023));
#61361=CARTESIAN_POINT('Ctrl Pts',(-18.0714612955843,-16.4792196892665,
-13.1999651227939));
#61362=CARTESIAN_POINT('Ctrl Pts',(-17.9862791665498,-16.5020427670648,
-13.2043515848065));
#61363=CARTESIAN_POINT('Ctrl Pts',(-17.9023749641123,-16.5292463408117,
-13.208738046819));
#61364=CARTESIAN_POINT('Ctrl Pts',(-17.8202171381046,-16.5606403697256,
-13.2131245088315));
#61365=CARTESIAN_POINT('Ctrl Pts',(-17.738059312097,-16.5920343986395,-13.2175109708441));
#61366=CARTESIAN_POINT('Ctrl Pts',(-17.6576483623232,-16.6276185783625,
-13.2218974328566));
#61367=CARTESIAN_POINT('Ctrl Pts',(-17.579422411398,-16.6671475776545,-13.2262838948691));
#61368=CARTESIAN_POINT('Ctrl Pts',(-17.5048157787117,-16.7048476694496,
-13.2304674063035));
#61369=CARTESIAN_POINT('Ctrl Pts',(-17.4319187998419,-16.746275904748,-13.2346509177379));
#61370=CARTESIAN_POINT('Ctrl Pts',(-17.3611287395177,-16.7912537163883,
-13.2388344291723));
#61371=CARTESIAN_POINT('Ctrl Pts',(-17.2970899771861,-16.8319419624025,
-13.2426189561699));
#61372=CARTESIAN_POINT('Ctrl Pts',(-17.2347754579772,-16.8755343097897,
-13.2464034831674));
#61373=CARTESIAN_POINT('Ctrl Pts',(-17.1744641548914,-16.9218650419685,
-13.250188010165));
#61374=CARTESIAN_POINT('Ctrl Pts',(-17.1725834092545,-16.9193794902115,
-12.4500366838548));
#61375=CARTESIAN_POINT('Ctrl Pts',(-17.1023021766235,-16.9725280716596,
-12.4544341408301));
#61376=CARTESIAN_POINT('Ctrl Pts',(-16.385846986399,-17.5778645097674,-12.5012235333658));
#61377=CARTESIAN_POINT('Ctrl Pts',(-15.7591749835997,-19.5120954830799,
-12.590404861462));
#61378=CARTESIAN_POINT('Ctrl Pts',(-17.5947353048798,-21.7565261244674,
-12.7175806681434));
#61379=CARTESIAN_POINT('Ctrl Pts',(-20.4360628533385,-21.4324759086211,
-12.8430154491812));
#61380=CARTESIAN_POINT('Ctrl Pts',(-21.2952859035193,-19.7651270969621,
-12.9260582946585));
#61381=CARTESIAN_POINT('Ctrl Pts',(-21.2980343668152,-18.9513691597422,
-12.9667092045753));
#61382=CARTESIAN_POINT('Origin',(-18.734,-18.952,1.76670989022851));
#61383=CARTESIAN_POINT('',(-17.1744641548914,-16.9218650419685,-11.6500725286462));
#61384=CARTESIAN_POINT('',(-17.1744641548914,-16.9218650419685,-11.716761786294));
#61385=CARTESIAN_POINT('',(-17.1744641548914,-16.9218650419685,1.76670989022851));
#61386=CARTESIAN_POINT('',(-21.2939989766127,-18.9542890482673,-12.2332901098107));
#61387=CARTESIAN_POINT('Ctrl Pts',(-17.1744641548914,-16.9218650419685,
-11.716761786294));
#61388=CARTESIAN_POINT('Ctrl Pts',(-17.1079832457044,-16.9729352235259,
-11.7209383110854));
#61389=CARTESIAN_POINT('Ctrl Pts',(-17.0439255031023,-17.0273420721353,
-11.7251148358768));
#61390=CARTESIAN_POINT('Ctrl Pts',(-16.9826416876458,-17.0848245766003,
-11.7292913606681));
#61391=CARTESIAN_POINT('Ctrl Pts',(-16.9214167468941,-17.1422518582393,
-11.7334638731168));
#61392=CARTESIAN_POINT('Ctrl Pts',(-16.8629607713186,-17.2027486100786,
-11.7376363855656));
#61393=CARTESIAN_POINT('Ctrl Pts',(-16.8075914573689,-17.2660136041837,
-11.7418088980143));
#61394=CARTESIAN_POINT('Ctrl Pts',(-16.7522504334316,-17.3292462741122,
-11.7459792785886));
#61395=CARTESIAN_POINT('Ctrl Pts',(-16.6999932422071,-17.3952440324702,
-11.7501496591628));
#61396=CARTESIAN_POINT('Ctrl Pts',(-16.6510998775129,-17.4636697007239,
-11.754320039737));
#61397=CARTESIAN_POINT('Ctrl Pts',(-16.6022168271016,-17.5320809342644,
-11.75848954055));
#61398=CARTESIAN_POINT('Ctrl Pts',(-16.5566964608029,-17.6029186859973,
-11.762659041363));
#61399=CARTESIAN_POINT('Ctrl Pts',(-16.5147768698912,-17.6758147866433,
-11.7668285421761));
#61400=CARTESIAN_POINT('Ctrl Pts',(-16.4728535473591,-17.7487173763933,
-11.7709984141519));
#61401=CARTESIAN_POINT('Ctrl Pts',(-16.4345318648703,-17.8236782794338,
-11.7751682861278));
#61402=CARTESIAN_POINT('Ctrl Pts',(-16.4000044799957,-17.9003037926285,
-11.7793381581037));
#61403=CARTESIAN_POINT('Ctrl Pts',(-16.3654406882584,-17.977010102401,-11.783512426936));
#61404=CARTESIAN_POINT('Ctrl Pts',(-16.3346793719312,-18.0553841066984,
-11.7876866957684));
#61405=CARTESIAN_POINT('Ctrl Pts',(-16.3078652231149,-18.1350116008238,
-11.7918609646007));
#61406=CARTESIAN_POINT('Ctrl Pts',(-16.2810362571641,-18.2146830960208,
-11.7960375400774));
#61407=CARTESIAN_POINT('Ctrl Pts',(-16.2581589268918,-18.2956090173988,
-11.800214115554));
#61408=CARTESIAN_POINT('Ctrl Pts',(-16.2393274875384,-18.3773618046384,
-11.8043906910306));
#61409=CARTESIAN_POINT('Ctrl Pts',(-16.220463547881,-18.459255685205,-11.8085744746643));
#61410=CARTESIAN_POINT('Ctrl Pts',(-16.2056595258686,-18.5419788285982,
-11.8127582582979));
#61411=CARTESIAN_POINT('Ctrl Pts',(-16.1949581528301,-18.6250955822875,
-11.8169420419316));
#61412=CARTESIAN_POINT('Ctrl Pts',(-16.1872902945174,-18.6846512569105,
-11.8199398497828));
#61413=CARTESIAN_POINT('Ctrl Pts',(-16.181727707034,-18.7444088772759,-11.8229376576341));
#61414=CARTESIAN_POINT('Ctrl Pts',(-16.1782696504242,-18.8042083214207,
-11.8259354654853));
#61415=CARTESIAN_POINT('Ctrl Pts',(-16.1734425556468,-18.8876822540642,
-11.8301200998784));
#61416=CARTESIAN_POINT('Ctrl Pts',(-16.172700351485,-18.9715482669721,-11.8343047342714));
#61417=CARTESIAN_POINT('Ctrl Pts',(-16.1760879473577,-19.0553727766261,
-11.8384893686645));
#61418=CARTESIAN_POINT('Ctrl Pts',(-16.179470721407,-19.1390779724659,-11.8426680467484));
#61419=CARTESIAN_POINT('Ctrl Pts',(-16.186971601001,-19.2227413266666,-11.8468467248323));
#61420=CARTESIAN_POINT('Ctrl Pts',(-16.1985835897661,-19.3059260187055,
-11.8510254029163));
#61421=CARTESIAN_POINT('Ctrl Pts',(-16.2104037150845,-19.3906017365655,
-11.8552789808017));
#61422=CARTESIAN_POINT('Ctrl Pts',(-16.2264838103271,-19.4747809821047,
-11.8595325586872));
#61423=CARTESIAN_POINT('Ctrl Pts',(-16.2467609749144,-19.5580049769523,
-11.8637861365726));
#61424=CARTESIAN_POINT('Ctrl Pts',(-16.2666450270985,-19.6396155122616,
-11.8679572505505));
#61425=CARTESIAN_POINT('Ctrl Pts',(-16.2905647501889,-19.7203070376072,
-11.8721283645285));
#61426=CARTESIAN_POINT('Ctrl Pts',(-16.3184090347921,-19.7996557607931,
-11.8762994785064));
#61427=CARTESIAN_POINT('Ctrl Pts',(-16.3462439759767,-19.8789778577487,
-11.8804691928268));
#61428=CARTESIAN_POINT('Ctrl Pts',(-16.3780007110438,-19.9569576137028,
-11.8846389071472));
#61429=CARTESIAN_POINT('Ctrl Pts',(-16.4135185064017,-20.0331871428518,
-11.8888086214675));
#61430=CARTESIAN_POINT('Ctrl Pts',(-16.4490350378841,-20.109413959427,-11.8929781874116));
#61431=CARTESIAN_POINT('Ctrl Pts',(-16.4883121684974,-20.1838902563955,
-11.8971477533556));
#61432=CARTESIAN_POINT('Ctrl Pts',(-16.531141898202,-20.2562301113465,-11.9013173192997));
#61433=CARTESIAN_POINT('Ctrl Pts',(-16.5754774683667,-20.3311133463566,
-11.9056334820386));
#61434=CARTESIAN_POINT('Ctrl Pts',(-16.6236198358017,-20.4037066556453,
-11.9099496447775));
#61435=CARTESIAN_POINT('Ctrl Pts',(-16.6752887227193,-20.4736135766998,
-11.9142658075164));
#61436=CARTESIAN_POINT('Ctrl Pts',(-16.7252745010802,-20.5412432871539,
-11.9184413717081));
#61437=CARTESIAN_POINT('Ctrl Pts',(-16.778560239593,-20.6063586052094,-11.9226169358998));
#61438=CARTESIAN_POINT('Ctrl Pts',(-16.8348515919043,-20.6686348837268,
-11.9267925000914));
#61439=CARTESIAN_POINT('Ctrl Pts',(-16.8939860866009,-20.7340565890242,
-11.931178962104));
#61440=CARTESIAN_POINT('Ctrl Pts',(-16.9564373882607,-20.7963445054469,
-11.9355654241165));
#61441=CARTESIAN_POINT('Ctrl Pts',(-17.0218228555023,-20.8551682599969,
-11.9399518861291));
#61442=CARTESIAN_POINT('Ctrl Pts',(-17.0872083227439,-20.9139920145469,
-11.9443383481416));
#61443=CARTESIAN_POINT('Ctrl Pts',(-17.1555274568808,-20.9693513010386,
-11.9487248101541));
#61444=CARTESIAN_POINT('Ctrl Pts',(-17.2263622218881,-21.0209679383717,
-11.9531112721667));
#61445=CARTESIAN_POINT('Ctrl Pts',(-17.2939377743552,-21.0702096177069,
-11.9572959065597));
#61446=CARTESIAN_POINT('Ctrl Pts',(-17.3640540780907,-21.1162287760929,
-11.9614805409527));
#61447=CARTESIAN_POINT('Ctrl Pts',(-17.4363708665884,-21.1587529612808,
-11.9656651753458));
#61448=CARTESIAN_POINT('Ctrl Pts',(-17.5085847210887,-21.2012166185545,
-11.9698438534297));
#61449=CARTESIAN_POINT('Ctrl Pts',(-17.5829924458174,-21.2401949526837,
-11.9740225315137));
#61450=CARTESIAN_POINT('Ctrl Pts',(-17.659222956839,-21.2754574038476,-11.9782012095976));
#61451=CARTESIAN_POINT('Ctrl Pts',(-17.7368198449848,-21.3113519091059,
-11.9824547874831));
#61452=CARTESIAN_POINT('Ctrl Pts',(-17.8163051194007,-21.3433957227619,
-11.9867083653685));
#61453=CARTESIAN_POINT('Ctrl Pts',(-17.8972589731891,-21.3713934062181,
-11.9909619432539));
#61454=CARTESIAN_POINT('Ctrl Pts',(-17.9766433785533,-21.3988482999474,
-11.9951330572319));
#61455=CARTESIAN_POINT('Ctrl Pts',(-18.0574394740936,-21.4224123904404,
-11.9993041712098));
#61456=CARTESIAN_POINT('Ctrl Pts',(-18.1392307762325,-21.4419497124358,
-12.0034752851878));
#61457=CARTESIAN_POINT('Ctrl Pts',(-18.2209946325099,-21.461480478494,-12.0076449995081));
#61458=CARTESIAN_POINT('Ctrl Pts',(-18.303752585081,-21.4769870528098,-12.0118147138285));
#61459=CARTESIAN_POINT('Ctrl Pts',(-18.3870746644898,-21.4883838060477,
-12.0159844281489));
#61460=CARTESIAN_POINT('Ctrl Pts',(-18.4703937789414,-21.4997801537403,
-12.0201539940929));
#61461=CARTESIAN_POINT('Ctrl Pts',(-18.5542765244138,-21.5070669096296,
-12.024323560037));
#61462=CARTESIAN_POINT('Ctrl Pts',(-18.6382858147563,-21.5102100763509,
-12.028493125981));
#61463=CARTESIAN_POINT('Ctrl Pts',(-18.7252487681107,-21.5134637529366,
-12.0328092887199));
#61464=CARTESIAN_POINT('Ctrl Pts',(-18.8123468034828,-21.5122770220956,
-12.0371254514589));
#61465=CARTESIAN_POINT('Ctrl Pts',(-18.8990948495902,-21.5066709554537,
-12.0414416141978));
#61466=CARTESIAN_POINT('Ctrl Pts',(-18.9830170872199,-21.501247505843,-12.0456171783895));
#61467=CARTESIAN_POINT('Ctrl Pts',(-19.0666113245951,-21.4916883190585,
-12.0497927425811));
#61468=CARTESIAN_POINT('Ctrl Pts',(-19.1494452607497,-21.4780651684627,
-12.0539683067728));
#61469=CARTESIAN_POINT('Ctrl Pts',(-19.2364629421006,-21.4637539449163,
-12.0583547687854));
#61470=CARTESIAN_POINT('Ctrl Pts',(-19.3226409276417,-21.444957551129,-12.0627412307979));
#61471=CARTESIAN_POINT('Ctrl Pts',(-19.4074943094419,-21.4218189033104,
-12.0671276928105));
#61472=CARTESIAN_POINT('Ctrl Pts',(-19.4923476912421,-21.3986802554918,
-12.071514154823));
#61473=CARTESIAN_POINT('Ctrl Pts',(-19.5758759419182,-21.371199607226,-12.0759006168356));
#61474=CARTESIAN_POINT('Ctrl Pts',(-19.6576188802164,-21.3395778865008,
-12.0802870788481));
#61475=CARTESIAN_POINT('Ctrl Pts',(-19.7356007047513,-21.3094111280209,
-12.0844717132412));
#61476=CARTESIAN_POINT('Ctrl Pts',(-19.8122481596154,-21.2753637103369,
-12.0886563476342));
#61477=CARTESIAN_POINT('Ctrl Pts',(-19.8871479757777,-21.2375742704974,
-12.0928409820272));
#61478=CARTESIAN_POINT('Ctrl Pts',(-19.9619411813225,-21.1998386192481,
-12.0970196601112));
#61479=CARTESIAN_POINT('Ctrl Pts',(-20.0349912820117,-21.1583717310105,
-12.1011983381951));
#61480=CARTESIAN_POINT('Ctrl Pts',(-20.1059035528267,-21.1133608309908,
-12.1053770162791));
#61481=CARTESIAN_POINT('Ctrl Pts',(-20.1780868751323,-21.0675431429372,
-12.1096305941645));
#61482=CARTESIAN_POINT('Ctrl Pts',(-20.2480545228573,-21.0180533145438,
-12.11388417205));
#61483=CARTESIAN_POINT('Ctrl Pts',(-20.3154149295588,-20.9651385497696,
-12.1181377499354));
#61484=CARTESIAN_POINT('Ctrl Pts',(-20.3814694233334,-20.9132496409652,
-12.1223088639134));
#61485=CARTESIAN_POINT('Ctrl Pts',(-20.4450164884367,-20.8580677061306,
-12.1264799778913));
#61486=CARTESIAN_POINT('Ctrl Pts',(-20.5057163649395,-20.7998693466275,
-12.1306510918693));
#61487=CARTESIAN_POINT('Ctrl Pts',(-20.5663958730126,-20.7416905161459,
-12.1348208061896));
#61488=CARTESIAN_POINT('Ctrl Pts',(-20.6242297581416,-20.6804975893352,
-12.13899052051));
#61489=CARTESIAN_POINT('Ctrl Pts',(-20.6789132852951,-20.6166057529285,
-12.1431602348304));
#61490=CARTESIAN_POINT('Ctrl Pts',(-20.7335948665741,-20.5527161900675,
-12.1473298007744));
#61491=CARTESIAN_POINT('Ctrl Pts',(-20.785126014285,-20.486128258616,-12.1514993667185));
#61492=CARTESIAN_POINT('Ctrl Pts',(-20.8332415555809,-20.4171910767277,
-12.1556689326625));
#61493=CARTESIAN_POINT('Ctrl Pts',(-20.8830487799517,-20.3458301485675,
-12.1599850954014));
#61494=CARTESIAN_POINT('Ctrl Pts',(-20.9291954417206,-20.2719521294864,
-12.1643012581404));
#61495=CARTESIAN_POINT('Ctrl Pts',(-20.9714366989051,-20.1959762933403,
-12.1686174208793));
#61496=CARTESIAN_POINT('Ctrl Pts',(-21.0123019515798,-20.1224753620654,
-12.172792985071));
#61497=CARTESIAN_POINT('Ctrl Pts',(-21.0495121634692,-20.0470116310055,
-12.1769685492626));
#61498=CARTESIAN_POINT('Ctrl Pts',(-21.0828936882991,-19.96998744642,-12.1811441134543));
#61499=CARTESIAN_POINT('Ctrl Pts',(-21.117961234591,-19.8890729533789,-12.1855305754669));
#61500=CARTESIAN_POINT('Ctrl Pts',(-21.1488029510882,-19.8064367740456,
-12.1899170374794));
#61501=CARTESIAN_POINT('Ctrl Pts',(-21.1752765362399,-19.7225639970856,
-12.1943034994919));
#61502=CARTESIAN_POINT('Ctrl Pts',(-21.2017501213916,-19.6386912201256,
-12.1986899615045));
#61503=CARTESIAN_POINT('Ctrl Pts',(-21.2238555029593,-19.5535824262448,
-12.203076423517));
#61504=CARTESIAN_POINT('Ctrl Pts',(-21.2415125421985,-19.4677333135615,
-12.2074628855296));
#61505=CARTESIAN_POINT('Ctrl Pts',(-21.2654843862316,-19.3511814097151,
-12.2134181072288));
#61506=CARTESIAN_POINT('Ctrl Pts',(-21.2813366135095,-19.2329068373031,
-12.219373328928));
#61507=CARTESIAN_POINT('Ctrl Pts',(-21.2888788650992,-19.1138455580776,
-12.2253285506272));
#61508=CARTESIAN_POINT('Ctrl Pts',(-21.2922399536332,-19.060787728371,-12.2279824036753));
#61509=CARTESIAN_POINT('Ctrl Pts',(-21.2939513313562,-19.0075739736056,
-12.2306362567234));
#61510=CARTESIAN_POINT('Ctrl Pts',(-21.293998976612,-18.9542890490546,-12.2332901097715));
#61511=CARTESIAN_POINT('Ctrl Pts',(-21.2939989766127,-18.9542890482673,
-12.2332901098107));
#61512=CARTESIAN_POINT('Ctrl Pts',(-21.2940747905549,-18.869501140071,-12.2375129674107));
#61513=CARTESIAN_POINT('Ctrl Pts',(-21.2899336304853,-18.7845778436852,
-12.2417358250107));
#61514=CARTESIAN_POINT('Ctrl Pts',(-21.2815646644669,-18.699979603286,-12.2459586826108));
#61515=CARTESIAN_POINT('Ctrl Pts',(-21.2734134565488,-18.6175825848873,
-12.2500716626647));
#61516=CARTESIAN_POINT('Ctrl Pts',(-21.2612518149667,-18.5354944186517,
-12.2541846427187));
#61517=CARTESIAN_POINT('Ctrl Pts',(-21.2451224198776,-18.4541403888767,
-12.2582976227727));
#61518=CARTESIAN_POINT('Ctrl Pts',(-21.2290007459443,-18.3728253033476,
-12.2624086339395));
#61519=CARTESIAN_POINT('Ctrl Pts',(-21.2089151790601,-18.2922441216167,
-12.2665196451063));
#61520=CARTESIAN_POINT('Ctrl Pts',(-21.1849598944702,-18.2128142346483,
-12.2706306562731));
#61521=CARTESIAN_POINT('Ctrl Pts',(-21.1610084101084,-18.1333969483105,
-12.2747410152756));
#61522=CARTESIAN_POINT('Ctrl Pts',(-21.133188564531,-18.0551310480641,-12.2788513742782));
#61523=CARTESIAN_POINT('Ctrl Pts',(-21.1016446063283,-17.9784194855459,
-12.2829617332807));
#61524=CARTESIAN_POINT('Ctrl Pts',(-21.0685960771622,-17.8980489659376,
-12.2872681465249));
#61525=CARTESIAN_POINT('Ctrl Pts',(-21.031459503672,-17.8193852938559,-12.2915745597691));
#61526=CARTESIAN_POINT('Ctrl Pts',(-20.9904568914618,-17.7428671301405,
-12.2958809730133));
#61527=CARTESIAN_POINT('Ctrl Pts',(-20.9512718262792,-17.669740832297,-12.2999964933321));
#61528=CARTESIAN_POINT('Ctrl Pts',(-20.9085564982552,-17.5985742591841,
-12.304112013651));
#61529=CARTESIAN_POINT('Ctrl Pts',(-20.8625501361326,-17.5297221375659,
-12.3082275339698));
#61530=CARTESIAN_POINT('Ctrl Pts',(-20.8165130556118,-17.4608240434608,
-12.3123458022171));
#61531=CARTESIAN_POINT('Ctrl Pts',(-20.7671808550883,-17.3942438526559,
-12.3164640704644));
#61532=CARTESIAN_POINT('Ctrl Pts',(-20.7148334041519,-17.3303036582036,
-12.3205823387118));
#61533=CARTESIAN_POINT('Ctrl Pts',(-20.6624054653519,-17.2662651512345,
-12.3247069390843));
#61534=CARTESIAN_POINT('Ctrl Pts',(-20.6069533520103,-17.204875081262,-12.3288315394568));
#61535=CARTESIAN_POINT('Ctrl Pts',(-20.5487934990227,-17.146418499235,-12.3329561398293));
#61536=CARTESIAN_POINT('Ctrl Pts',(-20.5408850965653,-17.1384697484523,
-12.3335169906232));
#61537=CARTESIAN_POINT('Ctrl Pts',(-20.5329266770602,-17.1305751748486,
-12.3340778414171));
#61538=CARTESIAN_POINT('Ctrl Pts',(-20.524919080494,-17.1227354354489,-12.334638692211));
#61539=CARTESIAN_POINT('Ctrl Pts',(-20.4651725946905,-17.0642413698601,
-12.338823326604));
#61540=CARTESIAN_POINT('Ctrl Pts',(-20.4024461555816,-17.0085686402269,
-12.3430079609971));
#61541=CARTESIAN_POINT('Ctrl Pts',(-20.3370370650427,-16.9560360303604,
-12.3471925953901));
#61542=CARTESIAN_POINT('Ctrl Pts',(-20.2717210762481,-16.9035781941619,
-12.3513712734741));
#61543=CARTESIAN_POINT('Ctrl Pts',(-20.2037303762193,-16.8542518853563,
-12.355549951558));
#61544=CARTESIAN_POINT('Ctrl Pts',(-20.1333988170805,-16.8083388908799,
-12.3597286296419));
#61545=CARTESIAN_POINT('Ctrl Pts',(-20.0618066152904,-16.7616029389746,
-12.3639822075274));
#61546=CARTESIAN_POINT('Ctrl Pts',(-19.9877891536757,-16.7184042096101,
-12.3682357854128));
#61547=CARTESIAN_POINT('Ctrl Pts',(-19.9117335730786,-16.6789967816029,
-12.3724893632982));
#61548=CARTESIAN_POINT('Ctrl Pts',(-19.8371524783216,-16.6403533434849,
-12.3766604772762));
#61549=CARTESIAN_POINT('Ctrl Pts',(-19.760612012467,-16.605355736394,-12.3808315912541));
#61550=CARTESIAN_POINT('Ctrl Pts',(-19.6825046263015,-16.5741987101768,
-12.3850027052321));
#61551=CARTESIAN_POINT('Ctrl Pts',(-19.6044234498237,-16.5430521390007,
-12.3891724195525));
#61552=CARTESIAN_POINT('Ctrl Pts',(-19.5247768242089,-16.5157437595369,
-12.3933421338728));
#61553=CARTESIAN_POINT('Ctrl Pts',(-19.443977821747,-16.4924204642607,-12.3975118481932));
#61554=CARTESIAN_POINT('Ctrl Pts',(-19.3631816944604,-16.4690979989275,
-12.4016814141372));
#61555=CARTESIAN_POINT('Ctrl Pts',(-19.2812337140819,-16.449760462599,-12.4058509800813));
#61556=CARTESIAN_POINT('Ctrl Pts',(-19.1985614595122,-16.4345046871273,
-12.4100205460253));
#61557=CARTESIAN_POINT('Ctrl Pts',(-19.1129825504589,-16.4187125374101,
-12.4143367087642));
#61558=CARTESIAN_POINT('Ctrl Pts',(-19.0266280073014,-16.4072946141391,
-12.4186528715032));
#61559=CARTESIAN_POINT('Ctrl Pts',(-18.9399808515253,-16.400300196182,-12.4229690342421));
#61560=CARTESIAN_POINT('Ctrl Pts',(-18.856156217735,-16.3935336206541,-12.4271445984338));
#61561=CARTESIAN_POINT('Ctrl Pts',(-18.7720582145667,-16.3909067522804,
-12.4313201626255));
#61562=CARTESIAN_POINT('Ctrl Pts',(-18.6881249777986,-16.3924110716097,
-12.4354957268171));
#61563=CARTESIAN_POINT('Ctrl Pts',(-18.5999524727736,-16.3939913705322,
-12.4398821888297));
#61564=CARTESIAN_POINT('Ctrl Pts',(-18.5119623987475,-16.4001311167978,
-12.4442686508422));
#61565=CARTESIAN_POINT('Ctrl Pts',(-18.4246552312345,-16.4107590011891,
-12.4486551128548));
#61566=CARTESIAN_POINT('Ctrl Pts',(-18.3373480637214,-16.4213868855804,
-12.4530415748673));
#61567=CARTESIAN_POINT('Ctrl Pts',(-18.2507243612256,-16.4365027334242,
-12.4574280368799));
#61568=CARTESIAN_POINT('Ctrl Pts',(-18.1652685194104,-16.4559742583486,
-12.4618144988924));
#61569=CARTESIAN_POINT('Ctrl Pts',(-18.0837368018554,-16.4745516526704,
-12.4659995349798));
#61570=CARTESIAN_POINT('Ctrl Pts',(-18.0029645350392,-16.49716262688,-12.4701845710671));
#61571=CARTESIAN_POINT('Ctrl Pts',(-17.9233808127844,-16.5237297239974,
-12.4743696071545));
#61572=CARTESIAN_POINT('Ctrl Pts',(-17.843930616112,-16.5502522468348,-12.4785476215876));
#61573=CARTESIAN_POINT('Ctrl Pts',(-17.7656654318456,-16.5807175510247,
-12.4827256360207));
#61574=CARTESIAN_POINT('Ctrl Pts',(-17.6890027069078,-16.6149975058999,
-12.4869036504538));
#61575=CARTESIAN_POINT('Ctrl Pts',(-17.6124142567096,-16.6492442486147,
-12.4910776170145));
#61576=CARTESIAN_POINT('Ctrl Pts',(-17.5374256012172,-16.6872981182065,
-12.4952515835751));
#61577=CARTESIAN_POINT('Ctrl Pts',(-17.4644368058942,-16.7289819397558,
-12.4994255501358));
#61578=CARTESIAN_POINT('Ctrl Pts',(-17.3915013099807,-16.7706353220704,
-12.503596468695));
#61579=CARTESIAN_POINT('Ctrl Pts',(-17.320563170554,-16.81591316144,-12.5077673872542));
#61580=CARTESIAN_POINT('Ctrl Pts',(-17.2519990079484,-16.8645917841596,
-12.5119383058134));
#61581=CARTESIAN_POINT('Ctrl Pts',(-17.2258010851161,-16.8831915708868,
-12.5135319868036));
#61582=CARTESIAN_POINT('Ctrl Pts',(-17.1999494849507,-16.9022873850278,
-12.5151256677938));
#61583=CARTESIAN_POINT('Ctrl Pts',(-17.1744641548914,-16.9218650419685,
-12.516719348784));
#61584=CARTESIAN_POINT('',(-21.2939992159918,-18.9499964727371,-12.1667098902285));
#61585=CARTESIAN_POINT('Ctrl Pts',(-21.2916488572292,-18.9499800095201,
-12.1667107986763));
#61586=CARTESIAN_POINT('Ctrl Pts',(-21.2937096036451,-18.6667985676303,
-12.1807663462568));
#61587=CARTESIAN_POINT('Ctrl Pts',(-21.1196059381089,-17.531999452779,-12.2372138293977));
#61588=CARTESIAN_POINT('Ctrl Pts',(-19.5298543213825,-16.0798455362524,
-12.3316557911239));
#61589=CARTESIAN_POINT('Ctrl Pts',(-17.7798204562966,-16.4601703038494,
-12.4120422052696));
#61590=CARTESIAN_POINT('Ctrl Pts',(-17.1725834092545,-16.9193794902115,
-12.4500366838548));
#61591=CARTESIAN_POINT('Ctrl Pts',(-17.1744641548914,-16.9218650419685,
-11.6500725286462));
#61592=CARTESIAN_POINT('Ctrl Pts',(-17.1077138142499,-16.9731421989338,
-11.65424766915));
#61593=CARTESIAN_POINT('Ctrl Pts',(-17.0435213657551,-17.0276947206701,
-11.6584228096539));
#61594=CARTESIAN_POINT('Ctrl Pts',(-16.9822122674274,-17.0852274535959,
-11.6625979501577));
#61595=CARTESIAN_POINT('Ctrl Pts',(-16.920893230811,-17.1427695126565,-11.6667737674575));
#61596=CARTESIAN_POINT('Ctrl Pts',(-16.8624587859411,-17.2032924040061,
-11.6709495847573));
#61597=CARTESIAN_POINT('Ctrl Pts',(-16.8071962002176,-17.2664653319661,
-11.6751254020571));
#61598=CARTESIAN_POINT('Ctrl Pts',(-16.7518333044684,-17.3297529284301,
-11.6793087991025));
#61599=CARTESIAN_POINT('Ctrl Pts',(-16.6996540596349,-17.3956998124642,
-11.6834921961479));
#61600=CARTESIAN_POINT('Ctrl Pts',(-16.6509044868842,-17.4639431854808,
-11.6876755931933));
#61601=CARTESIAN_POINT('Ctrl Pts',(-16.6023552296323,-17.5319061415721,
-11.6918418003595));
#61602=CARTESIAN_POINT('Ctrl Pts',(-16.5572076777017,-17.6021463237409,
-11.6960080075258));
#61603=CARTESIAN_POINT('Ctrl Pts',(-16.5156592733601,-17.6742815566288,
-11.700174214692));
#61604=CARTESIAN_POINT('Ctrl Pts',(-16.4739270995034,-17.7467358452539,
-11.704358849085));
#61605=CARTESIAN_POINT('Ctrl Pts',(-16.4356706929265,-17.8213716700561,
-11.7085434834781));
#61606=CARTESIAN_POINT('Ctrl Pts',(-16.4011245523601,-17.8978215778158,
-11.7127281178711));
#61607=CARTESIAN_POINT('Ctrl Pts',(-16.3666275839487,-17.9741626685944,
-11.7169067959551));
#61608=CARTESIAN_POINT('Ctrl Pts',(-16.3358305794285,-18.0523122977898,
-11.721085474039));
#61609=CARTESIAN_POINT('Ctrl Pts',(-16.3089230895031,-18.1318768518236,
-11.7252641521229));
#61610=CARTESIAN_POINT('Ctrl Pts',(-16.2815333021588,-18.2128675433065,
-11.7295177300084));
#61611=CARTESIAN_POINT('Ctrl Pts',(-16.258174080664,-18.2953239658201,-11.7337713078938));
#61612=CARTESIAN_POINT('Ctrl Pts',(-16.2389948450999,-18.3788078184222,
-11.7380248857792));
#61613=CARTESIAN_POINT('Ctrl Pts',(-16.2201874364424,-18.4606731736362,
-11.7421959997572));
#61614=CARTESIAN_POINT('Ctrl Pts',(-16.2053994934178,-18.5435260079657,
-11.7463671137351));
#61615=CARTESIAN_POINT('Ctrl Pts',(-16.194721659298,-18.6269376852946,-11.7505382277131));
#61616=CARTESIAN_POINT('Ctrl Pts',(-16.1840474082285,-18.7103213730297,
-11.7547079420335));
#61617=CARTESIAN_POINT('Ctrl Pts',(-16.1774805853424,-18.7942630754069,
-11.7588776563538));
#61618=CARTESIAN_POINT('Ctrl Pts',(-16.1750603443919,-18.8783261311159,
-11.7630473706742));
#61619=CARTESIAN_POINT('Ctrl Pts',(-16.172640189564,-18.9623861955006,-11.7672169366183));
#61620=CARTESIAN_POINT('Ctrl Pts',(-16.1743663356855,-19.0465671447644,
-11.7713865025623));
#61621=CARTESIAN_POINT('Ctrl Pts',(-16.1802258395509,-19.1304307636666,
-11.7755560685064));
#61622=CARTESIAN_POINT('Ctrl Pts',(-16.1862913563438,-19.2172429239522,
-11.7798722312453));
#61623=CARTESIAN_POINT('Ctrl Pts',(-16.1967862597982,-19.3037144978782,
-11.7841883939842));
#61624=CARTESIAN_POINT('Ctrl Pts',(-16.2116377216373,-19.3893654498161,
-11.7885045567231));
#61625=CARTESIAN_POINT('Ctrl Pts',(-16.2260053986691,-19.4722263310035,
-11.7926801209148));
#61626=CARTESIAN_POINT('Ctrl Pts',(-16.2444500136975,-19.5543187834628,
-11.7968556851065));
#61627=CARTESIAN_POINT('Ctrl Pts',(-16.2668539711946,-19.6352206616825,
-11.8010312492982));
#61628=CARTESIAN_POINT('Ctrl Pts',(-16.2903894993246,-19.7202087014451,
-11.8054177113107));
#61629=CARTESIAN_POINT('Ctrl Pts',(-16.3182946694535,-19.8038821804656,
-11.8098041733232));
#61630=CARTESIAN_POINT('Ctrl Pts',(-16.3503755250188,-19.8857742565901,
-11.8141906353358));
#61631=CARTESIAN_POINT('Ctrl Pts',(-16.382456380584,-19.9676663327146,-11.8185770973483));
#61632=CARTESIAN_POINT('Ctrl Pts',(-16.4187126130535,-20.0477765087051,
-11.8229635593609));
#61633=CARTESIAN_POINT('Ctrl Pts',(-16.4588952312817,-20.1256687315232,
-11.8273500213734));
#61634=CARTESIAN_POINT('Ctrl Pts',(-16.4972289876803,-20.1999770177056,
-11.8315346557664));
#61635=CARTESIAN_POINT('Ctrl Pts',(-16.5392784376738,-20.2725435578143,
-11.8357192901595));
#61636=CARTESIAN_POINT('Ctrl Pts',(-16.5848615409703,-20.3429722800687,
-11.8399039245525));
#61637=CARTESIAN_POINT('Ctrl Pts',(-16.6303797623612,-20.4133007557541,
-11.8440826026365));
#61638=CARTESIAN_POINT('Ctrl Pts',(-16.6794213986321,-20.4814970748824,
-11.8482612807204));
#61639=CARTESIAN_POINT('Ctrl Pts',(-16.7317580832551,-20.5471887997443,
-11.8524399588043));
#61640=CARTESIAN_POINT('Ctrl Pts',(-16.7850328653364,-20.6140580015628,
-11.8566935366898));
#61641=CARTESIAN_POINT('Ctrl Pts',(-16.8417217641061,-20.6783315077599,
-11.8609471145752));
#61642=CARTESIAN_POINT('Ctrl Pts',(-16.9015371160905,-20.7396464357065,
-11.8652006924607));
#61643=CARTESIAN_POINT('Ctrl Pts',(-16.9601928307565,-20.7997726541285,
-11.8693718064386));
#61644=CARTESIAN_POINT('Ctrl Pts',(-17.0218545195986,-20.8570536417638,
-11.8735429204166));
#61645=CARTESIAN_POINT('Ctrl Pts',(-17.0862108309602,-20.9111811693652,
-11.8777140343945));
#61646=CARTESIAN_POINT('Ctrl Pts',(-17.15054554694,-20.965290533952,-11.8818837487149));
#61647=CARTESIAN_POINT('Ctrl Pts',(-17.2175727378981,-21.0162482441934,
-11.8860534630352));
#61648=CARTESIAN_POINT('Ctrl Pts',(-17.2869464339592,-21.0637850214945,
-11.8902231773556));
#61649=CARTESIAN_POINT('Ctrl Pts',(-17.3563176614066,-21.1113201072332,
-11.8943927432997));
#61650=CARTESIAN_POINT('Ctrl Pts',(-17.42803484797,-21.155434242732,-11.8985623092437));
#61651=CARTESIAN_POINT('Ctrl Pts',(-17.5017225180692,-21.1959011135802,
-11.9027318751877));
#61652=CARTESIAN_POINT('Ctrl Pts',(-17.5780009557456,-21.237790749686,-11.9070480379267));
#61653=CARTESIAN_POINT('Ctrl Pts',(-17.6563905571824,-21.2757716196384,
-11.9113642006656));
#61654=CARTESIAN_POINT('Ctrl Pts',(-17.7364482678185,-21.3096451263118,
-11.9156803634045));
#61655=CARTESIAN_POINT('Ctrl Pts',(-17.8138981069511,-21.3424152070681,
-11.9198559275962));
#61656=CARTESIAN_POINT('Ctrl Pts',(-17.8929085883422,-21.3713412922625,
-11.9240314917879));
#61657=CARTESIAN_POINT('Ctrl Pts',(-17.9730611021937,-21.3962937617654,
-11.9282070559795));
#61658=CARTESIAN_POINT('Ctrl Pts',(-18.0572619289755,-21.4225065211841,
-11.9325935179921));
#61659=CARTESIAN_POINT('Ctrl Pts',(-18.142722622544,-21.4443335563954,-11.9369799800046));
#61660=CARTESIAN_POINT('Ctrl Pts',(-18.2289456575187,-21.4616852613706,
-11.9413664420172));
#61661=CARTESIAN_POINT('Ctrl Pts',(-18.3151686924933,-21.4790369663458,
-11.9457529040297));
#61662=CARTESIAN_POINT('Ctrl Pts',(-18.4021534837731,-21.4919133313661,
-11.9501393660423));
#61663=CARTESIAN_POINT('Ctrl Pts',(-18.489398605575,-21.500287691342,-11.9545258280548));
#61664=CARTESIAN_POINT('Ctrl Pts',(-18.5726294499945,-21.5082767346017,
-11.9587104624479));
#61665=CARTESIAN_POINT('Ctrl Pts',(-18.6564069960724,-21.5121986934545,
-11.9628950968409));
#61666=CARTESIAN_POINT('Ctrl Pts',(-18.7402996751639,-21.5119922488345,
-11.967079731234));
#61667=CARTESIAN_POINT('Ctrl Pts',(-18.8240729434106,-21.5117860980629,
-11.9712584093179));
#61668=CARTESIAN_POINT('Ctrl Pts',(-18.9079605630615,-21.507463217065,-11.9754370874019));
#61669=CARTESIAN_POINT('Ctrl Pts',(-18.9915257624726,-21.4990140324825,
-11.9796157654858));
#61670=CARTESIAN_POINT('Ctrl Pts',(-19.0765888080257,-21.4904134023388,
-11.9838693433712));
#61671=CARTESIAN_POINT('Ctrl Pts',(-19.1613172809486,-21.4775370395472,
-11.9881229212567));
#61672=CARTESIAN_POINT('Ctrl Pts',(-19.2452503475952,-21.4604304020809,
-11.9923764991421));
#61673=CARTESIAN_POINT('Ctrl Pts',(-19.3275562079629,-21.4436554101628,
-11.9965476131201));
#61674=CARTESIAN_POINT('Ctrl Pts',(-19.409096756315,-21.4228128002075,-12.000718727098));
#61675=CARTESIAN_POINT('Ctrl Pts',(-19.4894442918869,-21.3979975310404,
-12.004889841076));
#61676=CARTESIAN_POINT('Ctrl Pts',(-19.5697648660672,-21.3731905888764,
-12.0090595553963));
#61677=CARTESIAN_POINT('Ctrl Pts',(-19.6488927833422,-21.3444137706278,
-12.0132292697167));
#61678=CARTESIAN_POINT('Ctrl Pts',(-19.7264143560961,-21.3118122268126,
-12.0173989840371));
#61679=CARTESIAN_POINT('Ctrl Pts',(-19.8039331702998,-21.2792118431002,
-12.0215685499811));
#61680=CARTESIAN_POINT('Ctrl Pts',(-19.8798453299038,-21.242787183546,-12.0257381159252));
#61681=CARTESIAN_POINT('Ctrl Pts',(-19.9537573024934,-21.2027314639943,
-12.0299076818692));
#61682=CARTESIAN_POINT('Ctrl Pts',(-20.030267928859,-21.1612674347573,-12.0342238446082));
#61683=CARTESIAN_POINT('Ctrl Pts',(-20.1046346343673,-21.1159125099133,
-12.0385400073471));
#61684=CARTESIAN_POINT('Ctrl Pts',(-20.1764506132337,-21.0669317313762,
-12.042856170086));
#61685=CARTESIAN_POINT('Ctrl Pts',(-20.2459271941422,-21.019546496548,-12.0470317342777));
#61686=CARTESIAN_POINT('Ctrl Pts',(-20.3130163291632,-20.968768326667,-12.0512072984694));
#61687=CARTESIAN_POINT('Ctrl Pts',(-20.3773824427364,-20.914879045409,-12.0553828626611));
#61688=CARTESIAN_POINT('Ctrl Pts',(-20.4449995356903,-20.8582679446643,
-12.0597693246736));
#61689=CARTESIAN_POINT('Ctrl Pts',(-20.5096108706381,-20.7982235859986,
-12.0641557866861));
#61690=CARTESIAN_POINT('Ctrl Pts',(-20.5708718020379,-20.735115807478,-12.0685422486987));
#61691=CARTESIAN_POINT('Ctrl Pts',(-20.6321327334377,-20.6720080289574,
-12.0729287107112));
#61692=CARTESIAN_POINT('Ctrl Pts',(-20.6900429364135,-20.6058373172988,
-12.0773151727238));
#61693=CARTESIAN_POINT('Ctrl Pts',(-20.7443085775788,-20.5370108589259,
-12.0817016347363));
#61694=CARTESIAN_POINT('Ctrl Pts',(-20.796026764239,-20.4714154002739,-12.0858821780095));
#61695=CARTESIAN_POINT('Ctrl Pts',(-20.8446312405901,-20.4031588919979,
-12.0900627212828));
#61696=CARTESIAN_POINT('Ctrl Pts',(-20.8898359348525,-20.3325692383937,
-12.0942432645561));
#61697=CARTESIAN_POINT('Ctrl Pts',(-20.9349778718437,-20.2620775837717,
-12.0984180040186));
#61698=CARTESIAN_POINT('Ctrl Pts',(-20.9767291512524,-20.1892595981083,
-12.1025927434812));
#61699=CARTESIAN_POINT('Ctrl Pts',(-21.0148441174669,-20.114475854294,-12.1067674829437));
#61700=CARTESIAN_POINT('Ctrl Pts',(-21.0529176328921,-20.0397734392993,
-12.1109376822935));
#61701=CARTESIAN_POINT('Ctrl Pts',(-21.0873624809752,-19.9631099194739,
-12.1151078816433));
#61702=CARTESIAN_POINT('Ctrl Pts',(-21.1179772351408,-19.884873272385,-12.119278080993));
#61703=CARTESIAN_POINT('Ctrl Pts',(-21.1485693987593,-19.8066943559137,
-12.1234452031636));
#61704=CARTESIAN_POINT('Ctrl Pts',(-21.1753369141578,-19.7269450449952,
-12.1276123253341));
#61705=CARTESIAN_POINT('Ctrl Pts',(-21.1981256703524,-19.6460350716717,
-12.1317794475047));
#61706=CARTESIAN_POINT('Ctrl Pts',(-21.2209040463206,-19.5651619526563,
-12.1359446715606));
#61707=CARTESIAN_POINT('Ctrl Pts',(-21.2397071410259,-19.4831296648113,
-12.1401098956165));
#61708=CARTESIAN_POINT('Ctrl Pts',(-21.2544305326003,-19.4003636139743,
-12.1442751196725));
#61709=CARTESIAN_POINT('Ctrl Pts',(-21.2691564647156,-19.3175832817451,
-12.1484410624433));
#61710=CARTESIAN_POINT('Ctrl Pts',(-21.2798011983648,-19.2340693856731,
-12.1526070052142));
#61711=CARTESIAN_POINT('Ctrl Pts',(-21.2863115236391,-19.1502571216861,
-12.1567729479851));
#61712=CARTESIAN_POINT('Ctrl Pts',(-21.2914878410454,-19.0836185341096,
-12.1600852620662));
#61713=CARTESIAN_POINT('Ctrl Pts',(-21.2940514917317,-19.0167915973239,
-12.1633975761474));
#61714=CARTESIAN_POINT('Ctrl Pts',(-21.2939992159918,-18.9499964727371,
-12.1667098902285));
#61715=CARTESIAN_POINT('Origin',(-18.734,-18.952,1.76670989022851));
#61716=CARTESIAN_POINT('',(-17.1757181146141,-16.923465526843,-10.8502164882119));
#61717=CARTESIAN_POINT('',(-17.1731949518433,-16.9201829956178,-10.9165936692269));
#61718=CARTESIAN_POINT('',(-17.1744641548914,-16.9218650419685,1.76670989022851));
#61719=CARTESIAN_POINT('',(-21.2940195831445,-18.9506989550129,-11.4332901033027));
#61720=CARTESIAN_POINT('Ctrl Pts',(-17.1731949518433,-16.9201829956178,
-10.9165936692269));
#61721=CARTESIAN_POINT('Ctrl Pts',(-17.0711421091448,-16.9970800397133,
-10.9229640523897));
#61722=CARTESIAN_POINT('Ctrl Pts',(-16.3366273566849,-17.6446400359971,
-10.9717263711129));
#61723=CARTESIAN_POINT('Ctrl Pts',(-15.7882885392514,-19.6491907555867,
-11.0628806253967));
#61724=CARTESIAN_POINT('Ctrl Pts',(-17.7257693487527,-21.8062533022748,
-11.1900564320781));
#61725=CARTESIAN_POINT('Ctrl Pts',(-20.5048168108401,-21.3581664234228,
-11.3135258905536));
#61726=CARTESIAN_POINT('Ctrl Pts',(-21.2925956727874,-19.7256331618843,
-11.3946034134688));
#61727=CARTESIAN_POINT('Ctrl Pts',(-21.2974134759181,-18.9507193137797,
-11.4332890008234));
#61728=CARTESIAN_POINT('Ctrl Pts',(-21.2939996693303,-18.9506988355569,
-11.4332901097715));
#61729=CARTESIAN_POINT('Ctrl Pts',(-21.293961988618,-18.8765632322752,-11.436996088328));
#61730=CARTESIAN_POINT('Ctrl Pts',(-21.2907042434478,-18.8025118189363,
-11.4407020668845));
#61731=CARTESIAN_POINT('Ctrl Pts',(-21.2842464642989,-18.7287446051466,
-11.444408045441));
#61732=CARTESIAN_POINT('Ctrl Pts',(-21.2769546129518,-18.6454497843058,
-11.4485926798341));
#61733=CARTESIAN_POINT('Ctrl Pts',(-21.2655641024497,-18.5623575749322,
-11.4527773142271));
#61734=CARTESIAN_POINT('Ctrl Pts',(-21.250093180474,-18.4799034980303,-11.4569619486201));
#61735=CARTESIAN_POINT('Ctrl Pts',(-21.2346442794409,-18.3975667843011,
-11.4611406267041));
#61736=CARTESIAN_POINT('Ctrl Pts',(-21.2151265874821,-18.3158668471444,
-11.465319304788));
#61737=CARTESIAN_POINT('Ctrl Pts',(-21.1916101807317,-18.2352349062881,
-11.469497982872));
#61738=CARTESIAN_POINT('Ctrl Pts',(-21.1676722592913,-18.1531576958412,
-11.4737515607574));
#61739=CARTESIAN_POINT('Ctrl Pts',(-21.1395909011584,-18.07218762626,-11.4780051386429));
#61740=CARTESIAN_POINT('Ctrl Pts',(-21.1074946738889,-17.9927695620858,
-11.4822587165283));
#61741=CARTESIAN_POINT('Ctrl Pts',(-21.0760206946157,-17.9148911720574,
-11.4864298305062));
#61742=CARTESIAN_POINT('Ctrl Pts',(-21.0406863094724,-17.8385055933015,
-11.4906009444842));
#61743=CARTESIAN_POINT('Ctrl Pts',(-21.0016627302193,-17.7640161019717,
-11.4947720584621));
#61744=CARTESIAN_POINT('Ctrl Pts',(-20.962652245705,-17.6895516063101,-11.4989417727825));
#61745=CARTESIAN_POINT('Ctrl Pts',(-20.9199552389621,-17.6169823416316,
-11.5031114871029));
#61746=CARTESIAN_POINT('Ctrl Pts',(-20.8737897249261,-17.5466886704004,
-11.5072812014233));
#61747=CARTESIAN_POINT('Ctrl Pts',(-20.8276258536571,-17.4763975005198,
-11.5114507673673));
#61748=CARTESIAN_POINT('Ctrl Pts',(-20.7779939737416,-17.4083821471397,
-11.5156203333113));
#61749=CARTESIAN_POINT('Ctrl Pts',(-20.725155694621,-17.3429944065422,-11.5197898992554));
#61750=CARTESIAN_POINT('Ctrl Pts',(-20.6704596867895,-17.2753077136497,
-11.5241060619943));
#61751=CARTESIAN_POINT('Ctrl Pts',(-20.6123279420988,-17.2104372553888,
-11.5284222247332));
#61752=CARTESIAN_POINT('Ctrl Pts',(-20.5510951122123,-17.1487348078626,
-11.5327383874721));
#61753=CARTESIAN_POINT('Ctrl Pts',(-20.4918569353188,-17.0890423110747,
-11.5369139516638));
#61754=CARTESIAN_POINT('Ctrl Pts',(-20.4297169860238,-17.0323148814138,
-11.5410895158555));
#61755=CARTESIAN_POINT('Ctrl Pts',(-20.3650134540526,-16.9788312001506,
-11.5452650800472));
#61756=CARTESIAN_POINT('Ctrl Pts',(-20.2970419004996,-16.9226461852921,
-11.5496515420597));
#61757=CARTESIAN_POINT('Ctrl Pts',(-20.2262414538865,-16.8700415621995,
-11.5540380040722));
#61758=CARTESIAN_POINT('Ctrl Pts',(-20.1530384991427,-16.8212889126043,
-11.5584244660848));
#61759=CARTESIAN_POINT('Ctrl Pts',(-20.0798355443989,-16.7725362630091,
-11.5628109280973));
#61760=CARTESIAN_POINT('Ctrl Pts',(-20.0042306192382,-16.7276358177823,
-11.5671973901099));
#61761=CARTESIAN_POINT('Ctrl Pts',(-19.9266775857363,-16.6868023979171,
-11.5715838521224));
#61762=CARTESIAN_POINT('Ctrl Pts',(-19.852692882267,-16.6478477842295,-11.5757684865155));
#61763=CARTESIAN_POINT('Ctrl Pts',(-19.7766600165143,-16.6124491640088,
-11.5799531209085));
#61764=CARTESIAN_POINT('Ctrl Pts',(-19.6989550698441,-16.5808269331021,
-11.5841377553016));
#61765=CARTESIAN_POINT('Ctrl Pts',(-19.6213607265476,-16.549249712527,-11.5883164333855));
#61766=CARTESIAN_POINT('Ctrl Pts',(-19.5420994522192,-16.5214383763015,
-11.5924951114694));
#61767=CARTESIAN_POINT('Ctrl Pts',(-19.4615717652903,-16.4975674125468,
-11.5966737895534));
#61768=CARTESIAN_POINT('Ctrl Pts',(-19.3796006774474,-16.4732685789225,
-11.6009273674388));
#61769=CARTESIAN_POINT('Ctrl Pts',(-19.2963177561687,-16.4530529941954,
-11.6051809453242));
#61770=CARTESIAN_POINT('Ctrl Pts',(-19.2121666533115,-16.4370533501363,
-11.6094345232097));
#61771=CARTESIAN_POINT('Ctrl Pts',(-19.1296469837906,-16.4213638903979,
-11.6136056371876));
#61772=CARTESIAN_POINT('Ctrl Pts',(-19.0462929678283,-16.4097284515022,
-11.6177767511656));
#61773=CARTESIAN_POINT('Ctrl Pts',(-18.9625363705284,-16.4022213571869,
-11.6219478651435));
#61774=CARTESIAN_POINT('Ctrl Pts',(-18.8788078785636,-16.3947167819496,
-11.6261175794639));
#61775=CARTESIAN_POINT('Ctrl Pts',(-18.794677531367,-16.3913378410871,-11.6302872937843));
#61776=CARTESIAN_POINT('Ctrl Pts',(-18.7105831609267,-16.3921071015279,
-11.6344570081047));
#61777=CARTESIAN_POINT('Ctrl Pts',(-18.6264917829249,-16.3928763345952,
-11.6386265740487));
#61778=CARTESIAN_POINT('Ctrl Pts',(-18.54243683914,-16.3977934704174,-11.6427961399927));
#61779=CARTESIAN_POINT('Ctrl Pts',(-18.4588557388009,-16.4068289575101,
-11.6469657059368));
#61780=CARTESIAN_POINT('Ctrl Pts',(-18.3723360300824,-16.4161821211824,
-11.6512818686757));
#61781=CARTESIAN_POINT('Ctrl Pts',(-18.2863246298123,-16.4299485702282,
-11.6555980314146));
#61782=CARTESIAN_POINT('Ctrl Pts',(-18.2012984666217,-16.4480373252909,
-11.6599141941535));
#61783=CARTESIAN_POINT('Ctrl Pts',(-18.1190420217539,-16.46553684106,-11.6640897583452));
#61784=CARTESIAN_POINT('Ctrl Pts',(-18.0377080547433,-16.4870812228023,
-11.6682653225369));
#61785=CARTESIAN_POINT('Ctrl Pts',(-17.9577139481205,-16.5125369513646,
-11.6724408867286));
#61786=CARTESIAN_POINT('Ctrl Pts',(-17.8736795293402,-16.5392783882614,
-11.6768273487411));
#61787=CARTESIAN_POINT('Ctrl Pts',(-17.7911244272665,-16.570336474695,-11.6812138107537));
#61788=CARTESIAN_POINT('Ctrl Pts',(-17.7105077932321,-16.605499690457,-11.6856002727662));
#61789=CARTESIAN_POINT('Ctrl Pts',(-17.6298911591977,-16.640662906219,-11.6899867347788));
#61790=CARTESIAN_POINT('Ctrl Pts',(-17.5512134783828,-16.6799309241434,
-11.6943731967913));
#61791=CARTESIAN_POINT('Ctrl Pts',(-17.4749010481801,-16.7230383965788,
-11.6987596588038));
#61792=CARTESIAN_POINT('Ctrl Pts',(-17.4021059540752,-16.7641589912739,
-11.7029439432532));
#61793=CARTESIAN_POINT('Ctrl Pts',(-17.3311919413797,-16.8089259475395,
-11.7071282277026));
#61794=CARTESIAN_POINT('Ctrl Pts',(-17.2625477971695,-16.8571423879449,
-11.7113125121519));
#61795=CARTESIAN_POINT('Ctrl Pts',(-17.2327489339405,-16.8780734539456,
-11.713128936866));
#61796=CARTESIAN_POINT('Ctrl Pts',(-17.2033775631655,-16.8996539586958,
-11.71494536158));
#61797=CARTESIAN_POINT('Ctrl Pts',(-17.1744641548914,-16.9218650419685,
-11.716761786294));
#61798=CARTESIAN_POINT('',(-21.2939995125392,-18.9535798097909,-11.3667098902285));
#61799=CARTESIAN_POINT('Ctrl Pts',(-21.2939995125392,-18.9535798097909,
-11.3667098902285));
#61800=CARTESIAN_POINT('Ctrl Pts',(-21.2940518853803,-18.8687123476393,
-11.3709134538372));
#61801=CARTESIAN_POINT('Ctrl Pts',(-21.2898797137862,-18.7838299700766,
-11.3751170174459));
#61802=CARTESIAN_POINT('Ctrl Pts',(-21.2815050782104,-18.699377996817,-11.3793205810546));
#61803=CARTESIAN_POINT('Ctrl Pts',(-21.2731292177987,-18.6149136719984,
-11.3835247594572));
#61804=CARTESIAN_POINT('Ctrl Pts',(-21.2605497166712,-18.5308803238371,
-11.3877289378599));
#61805=CARTESIAN_POINT('Ctrl Pts',(-21.2438404672875,-18.4477175109462,
-11.3919331162626));
#61806=CARTESIAN_POINT('Ctrl Pts',(-21.2271240709727,-18.3645191274038,
-11.3961390928892));
#61807=CARTESIAN_POINT('Ctrl Pts',(-21.2062745049673,-18.2821924593938,
-11.4003450695159));
#61808=CARTESIAN_POINT('Ctrl Pts',(-21.1814163656274,-18.2011650425965,
-11.4045510461425));
#61809=CARTESIAN_POINT('Ctrl Pts',(-21.1565238219894,-18.1200254817903,
-11.408762843948));
#61810=CARTESIAN_POINT('Ctrl Pts',(-21.1276117659034,-18.0401891906194,
-11.4129746417534));
#61811=CARTESIAN_POINT('Ctrl Pts',(-21.0948539828413,-17.9620664306619,
-11.4171864395589));
#61812=CARTESIAN_POINT('Ctrl Pts',(-21.0620694457193,-17.8838798659899,
-11.4214016772397));
#61813=CARTESIAN_POINT('Ctrl Pts',(-21.0254331231614,-17.8074100228063,
-11.4256169149205));
#61814=CARTESIAN_POINT('Ctrl Pts',(-20.985165001354,-17.7330430127856,-11.4298321526013));
#61815=CARTESIAN_POINT('Ctrl Pts',(-20.9448260993907,-17.6585452862494,
-11.4340547994973));
#61816=CARTESIAN_POINT('Ctrl Pts',(-20.9008428915851,-17.5861581518394,
-11.4382774463933));
#61817=CARTESIAN_POINT('Ctrl Pts',(-20.853478708255,-17.5162388759777,-11.4425000932894));
#61818=CARTESIAN_POINT('Ctrl Pts',(-20.8410561777281,-17.497900666011,-11.4436075959693));
#61819=CARTESIAN_POINT('Ctrl Pts',(-20.828401284867,-17.4797320374709,-11.4447150986492));
#61820=CARTESIAN_POINT('Ctrl Pts',(-20.8155192213963,-17.4617390393097,
-11.4458226013291));
#61821=CARTESIAN_POINT('Ctrl Pts',(-20.766845094615,-17.3937535433782,-11.4500072357222));
#61822=CARTESIAN_POINT('Ctrl Pts',(-20.7147461245074,-17.3280286903786,
-11.4541918701152));
#61823=CARTESIAN_POINT('Ctrl Pts',(-20.6594597008471,-17.2649300724588,
-11.4583765045082));
#61824=CARTESIAN_POINT('Ctrl Pts',(-20.6042519705678,-17.2019212676116,
-11.4625551825922));
#61825=CARTESIAN_POINT('Ctrl Pts',(-20.5458660991116,-17.1415316158069,
-11.4667338606761));
#61826=CARTESIAN_POINT('Ctrl Pts',(-20.4845818988859,-17.0840966258147,
-11.4709125387601));
#61827=CARTESIAN_POINT('Ctrl Pts',(-20.4221992234154,-17.0256321549047,
-11.4751661166455));
#61828=CARTESIAN_POINT('Ctrl Pts',(-20.3568135727528,-16.9702297043271,
-11.479419694531));
#61829=CARTESIAN_POINT('Ctrl Pts',(-20.2887620518454,-16.9182067553113,
-11.4836732724164));
#61830=CARTESIAN_POINT('Ctrl Pts',(-20.2220298424625,-16.8671923726766,
-11.4878443863943));
#61831=CARTESIAN_POINT('Ctrl Pts',(-20.152734588911,-16.8194279167438,-11.4920155003723));
#61832=CARTESIAN_POINT('Ctrl Pts',(-20.081228933945,-16.7751733648401,-11.4961866143502));
#61833=CARTESIAN_POINT('Ctrl Pts',(-20.0097472733921,-16.7309336629788,
-11.5003563286706));
#61834=CARTESIAN_POINT('Ctrl Pts',(-19.9360570753463,-16.6902017679485,
-11.504526042991));
#61835=CARTESIAN_POINT('Ctrl Pts',(-19.8605396057917,-16.6531941107213,
-11.5086957573114));
#61836=CARTESIAN_POINT('Ctrl Pts',(-19.7850248234727,-16.6161877703852,
-11.5128653232554));
#61837=CARTESIAN_POINT('Ctrl Pts',(-19.7076833123969,-16.5829056060341,
-11.5170348891994));
#61838=CARTESIAN_POINT('Ctrl Pts',(-19.6289193227216,-16.5535172700602,
-11.5212044551435));
#61839=CARTESIAN_POINT('Ctrl Pts',(-19.5473860883352,-16.5230956764479,
-11.5255206178824));
#61840=CARTESIAN_POINT('Ctrl Pts',(-19.4643289796728,-16.4968470041692,
-11.5298367806213));
#61841=CARTESIAN_POINT('Ctrl Pts',(-19.3802151086562,-16.4749037093111,
-11.5341529433602));
#61842=CARTESIAN_POINT('Ctrl Pts',(-19.2988412381407,-16.453675214975,-11.5383285075519));
#61843=CARTESIAN_POINT('Ctrl Pts',(-19.2164788667992,-16.4364759603011,
-11.5425040717436));
#61844=CARTESIAN_POINT('Ctrl Pts',(-19.1335609462709,-16.4233736831601,
-11.5466796359353));
#61845=CARTESIAN_POINT('Ctrl Pts',(-19.0464550386954,-16.4096096411485,
-11.5510660979478));
#61846=CARTESIAN_POINT('Ctrl Pts',(-18.9587365661204,-16.4003673913993,
-11.5554525599604));
#61847=CARTESIAN_POINT('Ctrl Pts',(-18.8709107816371,-16.3956636688668,
-11.5598390219729));
#61848=CARTESIAN_POINT('Ctrl Pts',(-18.7830849971538,-16.3909599463343,
-11.5642254839854));
#61849=CARTESIAN_POINT('Ctrl Pts',(-18.6951524811212,-16.3907946760441,
-11.568611945998));
#61850=CARTESIAN_POINT('Ctrl Pts',(-18.607613246377,-16.3951217493771,-11.5729984080105));
#61851=CARTESIAN_POINT('Ctrl Pts',(-18.5241126314364,-16.3992491933198,
-11.577182500738));
#61852=CARTESIAN_POINT('Ctrl Pts',(-18.4406590445841,-16.4074789682953,
-11.5813665934654));
#61853=CARTESIAN_POINT('Ctrl Pts',(-18.3576882161454,-16.4198093592045,
-11.5855506861929));
#61854=CARTESIAN_POINT('Ctrl Pts',(-18.2748290034306,-16.4321231627717,
-11.5897291503091));
#61855=CARTESIAN_POINT('Ctrl Pts',(-18.1924517105566,-16.4485265622829,
-11.5939076144253));
#61856=CARTESIAN_POINT('Ctrl Pts',(-18.1109898384805,-16.4689659006281,
-11.5980860785415));
#61857=CARTESIAN_POINT('Ctrl Pts',(-18.0265307040886,-16.4901572724956,
-11.6024182827169));
#61858=CARTESIAN_POINT('Ctrl Pts',(-17.9430561635435,-16.5156873289273,
-11.6067504868923));
#61859=CARTESIAN_POINT('Ctrl Pts',(-17.8610409031935,-16.5454376352766,
-11.6110826910677));
#61860=CARTESIAN_POINT('Ctrl Pts',(-17.7820790639581,-16.5740803402701,
-11.6152536076529));
#61861=CARTESIAN_POINT('Ctrl Pts',(-17.7044702469478,-16.6066344546583,
-11.6194245242381));
#61862=CARTESIAN_POINT('Ctrl Pts',(-17.628623544901,-16.6429432894551,-11.6235954408233));
#61863=CARTESIAN_POINT('Ctrl Pts',(-17.5528073678039,-16.6792375115484,
-11.6277646787987));
#61864=CARTESIAN_POINT('Ctrl Pts',(-17.4787523097007,-16.7192832503609,
-11.631933916774));
#61865=CARTESIAN_POINT('Ctrl Pts',(-17.4068461498779,-16.7628762807676,
-11.6361031547494));
#61866=CARTESIAN_POINT('Ctrl Pts',(-17.3349387611569,-16.8064700561923,
-11.6402724639783));
#61867=CARTESIAN_POINT('Ctrl Pts',(-17.2651807378934,-16.853611006874,-11.6444417732072));
#61868=CARTESIAN_POINT('Ctrl Pts',(-17.1979329260742,-16.9040503071606,
-11.6486110824361));
#61869=CARTESIAN_POINT('Ctrl Pts',(-17.19007558454,-16.9099437154125,-11.6490982311728));
#61870=CARTESIAN_POINT('Ctrl Pts',(-17.1822524782037,-16.9158821050555,
-11.6495853799095));
#61871=CARTESIAN_POINT('Ctrl Pts',(-17.1744641548914,-16.9218650419685,
-11.6500725286462));
#61872=CARTESIAN_POINT('Ctrl Pts',(-17.1757181146138,-16.9234655268432,
-10.8502164882119));
#61873=CARTESIAN_POINT('Ctrl Pts',(-16.7160810052314,-17.2828444135616,
-10.8791841170091));
#61874=CARTESIAN_POINT('Ctrl Pts',(-15.8690425361355,-18.550019865754,-10.9505436813667));
#61875=CARTESIAN_POINT('Ctrl Pts',(-16.5533151791368,-21.0515010217726,
-11.0642951812848));
#61876=CARTESIAN_POINT('Ctrl Pts',(-19.3189847724962,-21.9220309163904,
-11.1914709879662));
#61877=CARTESIAN_POINT('Ctrl Pts',(-21.0857645353049,-20.4522478666649,
-11.2922755722919));
#61878=CARTESIAN_POINT('Ctrl Pts',(-21.2926071426957,-19.2766421748681,
-11.3506882210569));
#61879=CARTESIAN_POINT('Ctrl Pts',(-21.2907951752863,-18.9535971086061,
-11.3667089342616));
#61880=CARTESIAN_POINT('Origin',(-18.734,-18.952,1.76670989022851));
#61881=CARTESIAN_POINT('',(-17.1744641548914,-16.9218650419685,-10.0501312754282));
#61882=CARTESIAN_POINT('',(-17.1744641548914,-16.9218650419685,-10.1166694944115));
#61883=CARTESIAN_POINT('',(-17.1744641548914,-16.9218650419685,1.76670989022851));
#61884=CARTESIAN_POINT('',(-21.2939995125392,-18.9504201902087,-10.6332901097715));
#61885=CARTESIAN_POINT('Ctrl Pts',(-17.1744641548914,-16.9218650419685,
-10.1166694944115));
#61886=CARTESIAN_POINT('Ctrl Pts',(-17.1077744001828,-16.9730956572329,
-10.1208396545281));
#61887=CARTESIAN_POINT('Ctrl Pts',(-17.0436265325669,-17.0276044195277,
-10.1250098146447));
#61888=CARTESIAN_POINT('Ctrl Pts',(-16.9823480053276,-17.0851000858213,
-10.1291799747613));
#61889=CARTESIAN_POINT('Ctrl Pts',(-16.9210021848053,-17.1426588912327,
-10.1333547143575));
#61890=CARTESIAN_POINT('Ctrl Pts',(-16.8625323295411,-17.2032108319124,
-10.1375294539537));
#61891=CARTESIAN_POINT('Ctrl Pts',(-16.8072292042644,-17.2664276044321,
-10.1417041935499));
#61892=CARTESIAN_POINT('Ctrl Pts',(-16.7518918010427,-17.3296835599282,
-10.1458815207303));
#61893=CARTESIAN_POINT('Ctrl Pts',(-16.6997253198987,-17.3956072743516,
-10.1500588479107));
#61894=CARTESIAN_POINT('Ctrl Pts',(-16.6509788801178,-17.4638390496574,
-10.1542361750911));
#61895=CARTESIAN_POINT('Ctrl Pts',(-16.6021519993064,-17.5321834205567,
-10.1584203956673));
#61896=CARTESIAN_POINT('Ctrl Pts',(-16.5567566733308,-17.6028430682362,
-10.1626046162435));
#61897=CARTESIAN_POINT('Ctrl Pts',(-16.5149973069474,-17.6754315340627,
-10.1667888368197));
#61898=CARTESIAN_POINT('Ctrl Pts',(-16.4954988473035,-17.7093248469674,
-10.1687425507553));
#61899=CARTESIAN_POINT('Ctrl Pts',(-16.4767924206289,-17.7436383608983,
-10.170696264691));
#61900=CARTESIAN_POINT('Ctrl Pts',(-16.4588952312818,-17.7783312684767,
-10.1726499786266));
#61901=CARTESIAN_POINT('Ctrl Pts',(-16.4205614748832,-17.852639554659,-10.1768346130196));
#61902=CARTESIAN_POINT('Ctrl Pts',(-16.3858007370466,-17.9289661561368,
-10.1810192474127));
#61903=CARTESIAN_POINT('Ctrl Pts',(-16.3548302568731,-18.0069331593007,
-10.1852038818057));
#61904=CARTESIAN_POINT('Ctrl Pts',(-16.3239038593448,-18.0847891860857,
-10.1893825598897));
#61905=CARTESIAN_POINT('Ctrl Pts',(-16.2967571717625,-18.1642805528124,
-10.1935612379736));
#61906=CARTESIAN_POINT('Ctrl Pts',(-16.2735613224932,-18.2450052940591,
-10.1977399160575));
#61907=CARTESIAN_POINT('Ctrl Pts',(-16.2499497042962,-18.327176968277,-10.201993493943));
#61908=CARTESIAN_POINT('Ctrl Pts',(-16.2304321761498,-18.4106262399194,
-10.2062470718284));
#61909=CARTESIAN_POINT('Ctrl Pts',(-16.2151377103692,-18.4949083616214,
-10.2105006497138));
#61910=CARTESIAN_POINT('Ctrl Pts',(-16.2001397576524,-18.577556509931,-10.2146717636918));
#61911=CARTESIAN_POINT('Ctrl Pts',(-16.189202669843,-18.6610050301429,-10.2188428776697));
#61912=CARTESIAN_POINT('Ctrl Pts',(-16.1823971528001,-18.744821549959,-10.2230139916477));
#61913=CARTESIAN_POINT('Ctrl Pts',(-16.1755939194142,-18.8286099443324,
-10.2271837059681));
#61914=CARTESIAN_POINT('Ctrl Pts',(-16.1729195406043,-18.9127656349229,
-10.2313534202884));
#61915=CARTESIAN_POINT('Ctrl Pts',(-16.1743929164357,-18.9968506161326,
-10.2355231346088));
#61916=CARTESIAN_POINT('Ctrl Pts',(-16.175866239838,-19.0809326052378,-10.2396927005528));
#61917=CARTESIAN_POINT('Ctrl Pts',(-16.1814870155133,-19.1649434300175,
-10.2438622664969));
#61918=CARTESIAN_POINT('Ctrl Pts',(-16.1912220304802,-19.2484459440185,
-10.2480318324409));
#61919=CARTESIAN_POINT('Ctrl Pts',(-16.201299316564,-19.3348843034003,-10.2523479951798));
#61920=CARTESIAN_POINT('Ctrl Pts',(-16.2157854771196,-19.4207774186548,
-10.2566641579188));
#61921=CARTESIAN_POINT('Ctrl Pts',(-16.2345855425418,-19.5056491396623,
-10.2609803206577));
#61922=CARTESIAN_POINT('Ctrl Pts',(-16.2527731978103,-19.5877561732848,
-10.2651558848494));
#61923=CARTESIAN_POINT('Ctrl Pts',(-16.2749978531257,-19.6689068927544,
-10.269331449041));
#61924=CARTESIAN_POINT('Ctrl Pts',(-16.3011224991715,-19.7486850481605,
-10.2735070132327));
#61925=CARTESIAN_POINT('Ctrl Pts',(-16.3285666389836,-19.8324926085417,
-10.2778934752453));
#61926=CARTESIAN_POINT('Ctrl Pts',(-16.3603148903334,-19.9147847597323,
-10.2822799372578));
#61927=CARTESIAN_POINT('Ctrl Pts',(-16.3961518958429,-19.9951041376052,
-10.2866663992704));
#61928=CARTESIAN_POINT('Ctrl Pts',(-16.4319889013525,-20.0754235154782,
-10.2910528612829));
#61929=CARTESIAN_POINT('Ctrl Pts',(-16.4719143298048,-20.1537696376097,
-10.2954393232955));
#61930=CARTESIAN_POINT('Ctrl Pts',(-16.5156592733601,-20.2297184433711,
-10.299825785308));
#61931=CARTESIAN_POINT('Ctrl Pts',(-16.5573914472169,-20.3021727319963,
-10.3040104197011));
#61932=CARTESIAN_POINT('Ctrl Pts',(-16.6027547120117,-20.3727151532423,
-10.3081950540941));
#61933=CARTESIAN_POINT('Ctrl Pts',(-16.6515488896105,-20.4409584859349,
-10.3123796884872));
#61934=CARTESIAN_POINT('Ctrl Pts',(-16.7002736147369,-20.5091046826902,
-10.3165583665711));
#61935=CARTESIAN_POINT('Ctrl Pts',(-16.752419287262,-20.5749579200268,-10.3207370446551));
#61936=CARTESIAN_POINT('Ctrl Pts',(-16.807740546418,-20.6381567298107,-10.324915722739));
#61937=CARTESIAN_POINT('Ctrl Pts',(-16.8640533993856,-20.7024883328398,
-10.3291693006244));
#61938=CARTESIAN_POINT('Ctrl Pts',(-16.9236565628968,-20.7640689932945,
-10.3334228785099));
#61939=CARTESIAN_POINT('Ctrl Pts',(-16.9862458850687,-20.8225495325547,
-10.3376764563953));
#61940=CARTESIAN_POINT('Ctrl Pts',(-17.0476217910972,-20.8798963124459,
-10.3418475703733));
#61941=CARTESIAN_POINT('Ctrl Pts',(-17.1118687523879,-20.9342617737264,
-10.3460186843512));
#61942=CARTESIAN_POINT('Ctrl Pts',(-17.178661484003,-20.9853524290335,-10.3501897983292));
#61943=CARTESIAN_POINT('Ctrl Pts',(-17.2454318026719,-21.0364259403777,
-10.3543595126495));
#61944=CARTESIAN_POINT('Ctrl Pts',(-17.3147458300056,-21.0842265489049,
-10.3585292269699));
#61945=CARTESIAN_POINT('Ctrl Pts',(-17.3862455028589,-21.1285012785284,
-10.3626989412903));
#61946=CARTESIAN_POINT('Ctrl Pts',(-17.4577426314471,-21.1727744326672,
-10.3668685072343));
#61947=CARTESIAN_POINT('Ctrl Pts',(-17.5314248593523,-21.2135217158933,
-10.3710380731784));
#61948=CARTESIAN_POINT('Ctrl Pts',(-17.6069066380304,-21.2505344359839,
-10.3752076391224));
#61949=CARTESIAN_POINT('Ctrl Pts',(-17.6850422629298,-21.2888484776527,
-10.3795238018614));
#61950=CARTESIAN_POINT('Ctrl Pts',(-17.7651058639355,-21.3231602233056,
-10.3838399646003));
#61951=CARTESIAN_POINT('Ctrl Pts',(-17.8466456689033,-21.3532917963221,
-10.3881561273392));
#61952=CARTESIAN_POINT('Ctrl Pts',(-17.9255293233008,-21.382441836517,-10.3923316915309));
#61953=CARTESIAN_POINT('Ctrl Pts',(-18.0057940203934,-21.4076797638284,
-10.3965072557226));
#61954=CARTESIAN_POINT('Ctrl Pts',(-18.0870155993347,-21.4288954732277,
-10.4006828199143));
#61955=CARTESIAN_POINT('Ctrl Pts',(-18.1723394871422,-21.4511827376731,
-10.4050692819268));
#61956=CARTESIAN_POINT('Ctrl Pts',(-18.2587188895804,-21.469030663203,-10.4094557439393));
#61957=CARTESIAN_POINT('Ctrl Pts',(-18.345652666934,-21.4823727687636,-10.4138422059519));
#61958=CARTESIAN_POINT('Ctrl Pts',(-18.4325864442876,-21.4957148743243,
-10.4182286679644));
#61959=CARTESIAN_POINT('Ctrl Pts',(-18.5200740116329,-21.50455117729,-10.4226151299769));
#61960=CARTESIAN_POINT('Ctrl Pts',(-18.607613246377,-21.5088782506229,-10.4270015919895));
#61961=CARTESIAN_POINT('Ctrl Pts',(-18.6911246711665,-21.5130062288976,
-10.4311862263825));
#61962=CARTESIAN_POINT('Ctrl Pts',(-18.7749939587053,-21.5130461767751,
-10.4353708607756));
#61963=CARTESIAN_POINT('Ctrl Pts',(-18.8587871646378,-21.5089568169098,
-10.4395554951686));
#61964=CARTESIAN_POINT('Ctrl Pts',(-18.9424611013128,-21.5048732777422,
-10.4437341732526));
#61965=CARTESIAN_POINT('Ctrl Pts',(-19.0260587159289,-21.4966721277451,
-10.4479128513365));
#61966=CARTESIAN_POINT('Ctrl Pts',(-19.109143261859,-21.4843640206498,-10.4520915294204));
#61967=CARTESIAN_POINT('Ctrl Pts',(-19.1937170385632,-21.4718352995806,
-10.4563451073059));
#61968=CARTESIAN_POINT('Ctrl Pts',(-19.2777586906,-21.4550509150073,-10.4605986851913));
#61969=CARTESIAN_POINT('Ctrl Pts',(-19.3608099823631,-21.4340776067661,
-10.4648522630768));
#61970=CARTESIAN_POINT('Ctrl Pts',(-19.4422511627742,-21.4135109070312,
-10.4690233770547));
#61971=CARTESIAN_POINT('Ctrl Pts',(-19.5227395737971,-21.3889163729564,
-10.4731944910327));
#61972=CARTESIAN_POINT('Ctrl Pts',(-19.6018523684378,-21.3604086585538,
-10.4773656050106));
#61973=CARTESIAN_POINT('Ctrl Pts',(-19.6809386160161,-21.3319105101902,
-10.481535319331));
#61974=CARTESIAN_POINT('Ctrl Pts',(-19.7586497315282,-21.2995019451708,
-10.4857050336513));
#61975=CARTESIAN_POINT('Ctrl Pts',(-19.8345791893306,-21.2633471067783,
-10.4898747479717));
#61976=CARTESIAN_POINT('Ctrl Pts',(-19.9105059452373,-21.22719355493,-10.4940443139158));
#61977=CARTESIAN_POINT('Ctrl Pts',(-19.9846507545042,-21.1872941933041,
-10.4982138798598));
#61978=CARTESIAN_POINT('Ctrl Pts',(-20.0566294498838,-21.1438602460696,
-10.5023834458039));
#61979=CARTESIAN_POINT('Ctrl Pts',(-20.1311388273975,-21.0988992148319,
-10.5066996085428));
#61980=CARTESIAN_POINT('Ctrl Pts',(-20.2033264842381,-21.0501506938738,
-10.5110157712817));
#61981=CARTESIAN_POINT('Ctrl Pts',(-20.2727983186246,-20.9978982708332,
-10.5153319340206));
#61982=CARTESIAN_POINT('Ctrl Pts',(-20.3400071153131,-20.9473479649771,
-10.5195074982123));
#61983=CARTESIAN_POINT('Ctrl Pts',(-20.4046739763892,-20.8935188682645,
-10.523683062404));
#61984=CARTESIAN_POINT('Ctrl Pts',(-20.466476730727,-20.8367080350785,-10.5278586265957));
#61985=CARTESIAN_POINT('Ctrl Pts',(-20.5314009952643,-20.7770278217633,
-10.5322450886082));
#61986=CARTESIAN_POINT('Ctrl Pts',(-20.5931638083644,-20.7140571577261,
-10.5366315506207));
#61987=CARTESIAN_POINT('Ctrl Pts',(-20.651438012559,-20.6481814372272,-10.5410180126333));
#61988=CARTESIAN_POINT('Ctrl Pts',(-20.7097122167535,-20.5823057167282,
-10.5454044746458));
#61989=CARTESIAN_POINT('Ctrl Pts',(-20.7644975100435,-20.513525441,-10.5497909366584));
#61990=CARTESIAN_POINT('Ctrl Pts',(-20.8155192213965,-20.4422609606901,
-10.5541773986709));
#61991=CARTESIAN_POINT('Ctrl Pts',(-20.8646271615163,-20.3736695367859,
-10.5583993290636));
#61992=CARTESIAN_POINT('Ctrl Pts',(-20.9104308246501,-20.302523084569,-10.5626212594563));
#61993=CARTESIAN_POINT('Ctrl Pts',(-20.9526566798058,-20.2291697370174,
-10.5668431898491));
#61994=CARTESIAN_POINT('Ctrl Pts',(-20.9948201353165,-20.1559247880485,
-10.5710588812454));
#61995=CARTESIAN_POINT('Ctrl Pts',(-21.0334160638335,-20.0804798079433,
-10.5752745726417));
#61996=CARTESIAN_POINT('Ctrl Pts',(-21.0682129788551,-20.003213474678,-10.5794902640381));
#61997=CARTESIAN_POINT('Ctrl Pts',(-21.1029682787105,-19.9260395476302,
-10.583700913703));
#61998=CARTESIAN_POINT('Ctrl Pts',(-21.1339334100815,-19.8470490030809,
-10.587911563368));
#61999=CARTESIAN_POINT('Ctrl Pts',(-21.1609223976385,-19.7666457364035,
-10.592122213033));
#62000=CARTESIAN_POINT('Ctrl Pts',(-21.1878844462892,-19.6863227237952,
-10.5963286598616));
#62001=CARTESIAN_POINT('Ctrl Pts',(-21.2108781024615,-19.6045902181226,
-10.6005351066903));
#62002=CARTESIAN_POINT('Ctrl Pts',(-21.2297657078558,-19.5218715043685,
-10.6047415535189));
#62003=CARTESIAN_POINT('Ctrl Pts',(-21.24864245849,-19.4392003292924,-10.6089455828907));
#62004=CARTESIAN_POINT('Ctrl Pts',(-21.2634177498248,-19.3555445100527,
-10.6131496122625));
#62005=CARTESIAN_POINT('Ctrl Pts',(-21.27400421321,-19.2713408788045,-10.6173536416343));
#62006=CARTESIAN_POINT('Ctrl Pts',(-21.2845883389273,-19.1871558411237,
-10.6215567426863));
#62007=CARTESIAN_POINT('Ctrl Pts',(-21.2909854180498,-19.1024236771956,
-10.6257598437382));
#62008=CARTESIAN_POINT('Ctrl Pts',(-21.2931596531403,-19.0175886403171,
-10.6299629447901));
#62009=CARTESIAN_POINT('Ctrl Pts',(-21.2937333596144,-18.99520356793,-10.6310719997839));
#62010=CARTESIAN_POINT('Ctrl Pts',(-21.2940133304248,-18.9728113543426,
-10.6321810547777));
#62011=CARTESIAN_POINT('Ctrl Pts',(-21.2939995125392,-18.9504201902087,
-10.6332901097715));
#62012=CARTESIAN_POINT('Ctrl Pts',(-21.2907951936029,-18.9504028914923,
-10.633291065733));
#62013=CARTESIAN_POINT('Ctrl Pts',(-21.2926071610387,-18.6273578228792,
-10.6493117789394));
#62014=CARTESIAN_POINT('Ctrl Pts',(-21.0857645521851,-17.4517521226135,
-10.7077244277063));
#62015=CARTESIAN_POINT('Ctrl Pts',(-19.4306370810863,-16.0748525489571,
-10.802158628871));
#62016=CARTESIAN_POINT('Ctrl Pts',(-17.7502562881359,-16.4853659944509,
-10.8805721168292));
#62017=CARTESIAN_POINT('Ctrl Pts',(-17.1731949518433,-16.9201829956178,
-10.9165936692269));
#62018=CARTESIAN_POINT('',(-21.2940195635259,-18.9533010451044,-10.566709896691));
#62019=CARTESIAN_POINT('Ctrl Pts',(-21.2974134575541,-18.9532806863302,
-10.5667109991706));
#62020=CARTESIAN_POINT('Ctrl Pts',(-21.2925956544959,-18.178366843738,-10.6053965865272));
#62021=CARTESIAN_POINT('Ctrl Pts',(-20.5048167981983,-16.5458335938225,
-10.6864741094444));
#62022=CARTESIAN_POINT('Ctrl Pts',(-18.3777720107911,-16.2028740463623,
-10.7809759391248));
#62023=CARTESIAN_POINT('Ctrl Pts',(-17.3887251784425,-16.7569205723577,
-10.8367921814486));
#62024=CARTESIAN_POINT('Ctrl Pts',(-17.1757181146138,-16.9234655268432,
-10.8502164882119));
#62025=CARTESIAN_POINT('Ctrl Pts',(-17.1744641548914,-16.9218650419685,
-10.0501312754282));
#62026=CARTESIAN_POINT('Ctrl Pts',(-17.1081215409048,-16.972828986095,-10.0543142385325));
#62027=CARTESIAN_POINT('Ctrl Pts',(-17.0441627240079,-17.0271382362881,
-10.0584972016367));
#62028=CARTESIAN_POINT('Ctrl Pts',(-16.9829439471694,-17.084541111605,-10.0626801647409));
#62029=CARTESIAN_POINT('Ctrl Pts',(-16.9218070707038,-17.1418671915801,
-10.0668575317478));
#62030=CARTESIAN_POINT('Ctrl Pts',(-16.8634032855558,-17.2022783629591,
-10.0710348987546));
#62031=CARTESIAN_POINT('Ctrl Pts',(-16.8080570528915,-17.2654817627778,
-10.0752122657615));
#62032=CARTESIAN_POINT('Ctrl Pts',(-16.7527684355283,-17.3286193680025,
-10.0793852841388));
#62033=CARTESIAN_POINT('Ctrl Pts',(-16.7005313462713,-17.3945430800416,
-10.0835583025162));
#62034=CARTESIAN_POINT('Ctrl Pts',(-16.6516335517556,-17.4629231130576,
-10.0877313208936));
#62035=CARTESIAN_POINT('Ctrl Pts',(-16.6027633272263,-17.5312645914395,
-10.0919019864029));
#62036=CARTESIAN_POINT('Ctrl Pts',(-16.5572289263105,-17.6020592677418,
-10.0960726519122));
#62037=CARTESIAN_POINT('Ctrl Pts',(-16.515277225619,-17.6749450871466,-10.1002433174215));
#62038=CARTESIAN_POINT('Ctrl Pts',(-16.4733365938618,-17.7478116756661,
-10.1044128825029));
#62039=CARTESIAN_POINT('Ctrl Pts',(-16.4349770140236,-17.8227679128389,
-10.1085824475843));
#62040=CARTESIAN_POINT('Ctrl Pts',(-16.4004007511752,-17.8994248027412,
-10.1127520126657));
#62041=CARTESIAN_POINT('Ctrl Pts',(-16.3658232392718,-17.9760844618461,
-10.1169217283712));
#62042=CARTESIAN_POINT('Ctrl Pts',(-16.335029503705,-18.0544444757753,-10.1210914440766));
#62043=CARTESIAN_POINT('Ctrl Pts',(-16.3081741883135,-18.1340946684636,
-10.125261159782));
#62044=CARTESIAN_POINT('Ctrl Pts',(-16.2812914154966,-18.213826297143,-10.1294351386904));
#62045=CARTESIAN_POINT('Ctrl Pts',(-16.2583552528147,-18.2948503023518,
-10.1336091175987));
#62046=CARTESIAN_POINT('Ctrl Pts',(-16.2394706734754,-18.3767405462675,
-10.137783096507));
#62047=CARTESIAN_POINT('Ctrl Pts',(-16.2205765545129,-18.4586721573776,
-10.141959183918));
#62048=CARTESIAN_POINT('Ctrl Pts',(-16.2057381766318,-18.5414704255045,
-10.146135271329));
#62049=CARTESIAN_POINT('Ctrl Pts',(-16.1950090364198,-18.6247006158602,
-10.15031135874));
#62050=CARTESIAN_POINT('Ctrl Pts',(-16.1842607815537,-18.7080790861592,
-10.1544948861196));
#62051=CARTESIAN_POINT('Ctrl Pts',(-16.177636427472,-18.7918905566104,-10.1586784134992));
#62052=CARTESIAN_POINT('Ctrl Pts',(-16.1751373938136,-18.875696902679,-10.1628619408788));
#62053=CARTESIAN_POINT('Ctrl Pts',(-16.1729067675168,-18.9505020733664,
-10.1665961387575));
#62054=CARTESIAN_POINT('Ctrl Pts',(-16.1739621469759,-19.0253029292838,
-10.1703303366361));
#62055=CARTESIAN_POINT('Ctrl Pts',(-16.1782696504243,-19.0997916785801,
-10.1740645345148));
#62056=CARTESIAN_POINT('Ctrl Pts',(-16.1830967452018,-19.1832656112237,
-10.1782491689078));
#62057=CARTESIAN_POINT('Ctrl Pts',(-16.1920266966377,-19.2666581465938,
-10.1824338033009));
#62058=CARTESIAN_POINT('Ctrl Pts',(-16.205054135763,-19.3495334146438,-10.1866184376939));
#62059=CARTESIAN_POINT('Ctrl Pts',(-16.2180630319411,-19.4322907200076,
-10.1907971157779));
#62060=CARTESIAN_POINT('Ctrl Pts',(-16.235157760266,-19.514531769942,-10.1949757938618));
#62061=CARTESIAN_POINT('Ctrl Pts',(-16.2562810188397,-19.595823462137,-10.1991544719458));
#62062=CARTESIAN_POINT('Ctrl Pts',(-16.2777828966423,-19.6785722494913,
-10.2034080498312));
#62063=CARTESIAN_POINT('Ctrl Pts',(-16.3034591202046,-19.7603368285348,
-10.2076616277166));
#62064=CARTESIAN_POINT('Ctrl Pts',(-16.3331943249928,-19.840668729535,-10.2119152056021));
#62065=CARTESIAN_POINT('Ctrl Pts',(-16.3623530548127,-19.9194432398795,
-10.21608631958));
#62066=CARTESIAN_POINT('Ctrl Pts',(-16.3954146207213,-19.9968396756824,
-10.220257433558));
#62067=CARTESIAN_POINT('Ctrl Pts',(-16.4322198035646,-20.0724498771911,
-10.2244285475359));
#62068=CARTESIAN_POINT('Ctrl Pts',(-16.4690126360733,-20.1480347069665,
-10.2285982618563));
#62069=CARTESIAN_POINT('Ctrl Pts',(-16.5095463894923,-20.2218340795556,
-10.2327679761767));
#62070=CARTESIAN_POINT('Ctrl Pts',(-16.5536143847776,-20.2934613557352,
-10.236937690497));
#62071=CARTESIAN_POINT('Ctrl Pts',(-16.5976808119344,-20.365086083109,-10.2411072564411));
#62072=CARTESIAN_POINT('Ctrl Pts',(-16.6452809891204,-20.4345384763812,
-10.2452768223851));
#62073=CARTESIAN_POINT('Ctrl Pts',(-16.6961638176234,-20.5014591617066,
-10.2494463883292));
#62074=CARTESIAN_POINT('Ctrl Pts',(-16.7488356236058,-20.5707326957725,
-10.2537625510681));
#62075=CARTESIAN_POINT('Ctrl Pts',(-16.805024892642,-20.6372927599322,-10.258078713807));
#62076=CARTESIAN_POINT('Ctrl Pts',(-16.8644075151043,-20.7007778419289,
-10.2623948765459));
#62077=CARTESIAN_POINT('Ctrl Pts',(-16.9218557548858,-20.762194904057,-10.2665704407376));
#62078=CARTESIAN_POINT('Ctrl Pts',(-16.9822921248587,-20.820733948795,-10.2707460049293));
#62079=CARTESIAN_POINT('Ctrl Pts',(-17.0453868187422,-20.8761064222341,
-10.274921569121));
#62080=CARTESIAN_POINT('Ctrl Pts',(-17.1116682756204,-20.934275627671,-10.2793080311335));
#62081=CARTESIAN_POINT('Ctrl Pts',(-17.1808831995725,-20.9889496060668,
-10.283694493146));
#62082=CARTESIAN_POINT('Ctrl Pts',(-17.2526134178258,-21.0398442935608,
-10.2880809551586));
#62083=CARTESIAN_POINT('Ctrl Pts',(-17.3243436360791,-21.0907389810547,
-10.2924674171711));
#62084=CARTESIAN_POINT('Ctrl Pts',(-17.3985886179774,-21.1378541309858,
-10.2968538791837));
#62085=CARTESIAN_POINT('Ctrl Pts',(-17.4749010481802,-21.1809616034213,
-10.3012403411962));
#62086=CARTESIAN_POINT('Ctrl Pts',(-17.5477022303472,-21.2220856371494,
-10.3054249755892));
#62087=CARTESIAN_POINT('Ctrl Pts',(-17.6226557687809,-21.2597157589185,
-10.3096096099823));
#62088=CARTESIAN_POINT('Ctrl Pts',(-17.6993922596291,-21.2936205549928,
-10.3137942443753));
#62089=CARTESIAN_POINT('Ctrl Pts',(-17.7760195255806,-21.3274770917864,
-10.3179729224593));
#62090=CARTESIAN_POINT('Ctrl Pts',(-17.8544242858621,-21.3576186510691,
-10.3221516005432));
#62091=CARTESIAN_POINT('Ctrl Pts',(-17.9342113535405,-21.383858984603,-10.3263302786272));
#62092=CARTESIAN_POINT('Ctrl Pts',(-18.0154285470652,-21.410569657257,-10.3305838565126));
#62093=CARTESIAN_POINT('Ctrl Pts',(-18.0980776713418,-21.4332376324399,
-10.334837434398));
#62094=CARTESIAN_POINT('Ctrl Pts',(-18.1817191896631,-21.4517171653076,
-10.3390910122835));
#62095=CARTESIAN_POINT('Ctrl Pts',(-18.2637391539388,-21.4698384363709,
-10.3432621262614));
#62096=CARTESIAN_POINT('Ctrl Pts',(-18.3467129067617,-21.4839321143086,
-10.3474332402394));
#62097=CARTESIAN_POINT('Ctrl Pts',(-18.4302110680643,-21.4939111480997,
-10.3516043542173));
#62098=CARTESIAN_POINT('Ctrl Pts',(-18.5136812107525,-21.5038868333295,
-10.3557740685377));
#62099=CARTESIAN_POINT('Ctrl Pts',(-18.5976749560383,-21.5097505619763,
-10.3599437828581));
#62100=CARTESIAN_POINT('Ctrl Pts',(-18.6817553300755,-21.5114668379302,
-10.3641134971784));
#62101=CARTESIAN_POINT('Ctrl Pts',(-18.7658327121721,-21.5131830528116,
-10.3682830631225));
#62102=CARTESIAN_POINT('Ctrl Pts',(-18.8499962569365,-21.510752099899,-10.3724526290665));
#62103=CARTESIAN_POINT('Ctrl Pts',(-18.9338078728666,-21.5041905912256,
-10.3766221950106));
#62104=CARTESIAN_POINT('Ctrl Pts',(-19.02056620182,-21.4973983880017,-10.3809383577495));
#62105=CARTESIAN_POINT('Ctrl Pts',(-19.1069468680352,-21.4861798052051,
-10.3852545204884));
#62106=CARTESIAN_POINT('Ctrl Pts',(-19.1924704625208,-21.4706116880131,
-10.3895706832273));
#62107=CARTESIAN_POINT('Ctrl Pts',(-19.2752081349115,-21.4555507006011,
-10.393746247419));
#62108=CARTESIAN_POINT('Ctrl Pts',(-19.3571432683313,-21.4364193523527,
-10.3979218116107));
#62109=CARTESIAN_POINT('Ctrl Pts',(-19.4378547167233,-21.4133387693989,
-10.4020973758024));
#62110=CARTESIAN_POINT('Ctrl Pts',(-19.5226427085004,-21.3890924410691,
-10.4064838378149));
#62111=CARTESIAN_POINT('Ctrl Pts',(-19.6060795975569,-21.3604876310562,
-10.4108702998275));
#62112=CARTESIAN_POINT('Ctrl Pts',(-19.6877001821498,-21.3277221981047,
-10.41525676184));
#62113=CARTESIAN_POINT('Ctrl Pts',(-19.7693207667426,-21.2949567651532,
-10.4196432238525));
#62114=CARTESIAN_POINT('Ctrl Pts',(-19.8491245522346,-21.2580310219481,
-10.4240296858651));
#62115=CARTESIAN_POINT('Ctrl Pts',(-19.9266775857364,-21.2171976020829,
-10.4284161478776));
#62116=CARTESIAN_POINT('Ctrl Pts',(-20.0006622892057,-21.1782429883953,
-10.4326007822707));
#62117=CARTESIAN_POINT('Ctrl Pts',(-20.0728741952655,-21.1355873954291,
-10.4367854166637));
#62118=CARTESIAN_POINT('Ctrl Pts',(-20.1429187702871,-21.0894161734984,
-10.4409700510568));
#62119=CARTESIAN_POINT('Ctrl Pts',(-20.212863645526,-21.0433106705873,-10.4451487291407));
#62120=CARTESIAN_POINT('Ctrl Pts',(-20.2806469365542,-20.9936997293726,
-10.4493274072247));
#62121=CARTESIAN_POINT('Ctrl Pts',(-20.3458981308864,-20.9408148268869,
-10.4535060853086));
#62122=CARTESIAN_POINT('Ctrl Pts',(-20.4123189059818,-20.8869820005318,
-10.4577596631941));
#62123=CARTESIAN_POINT('Ctrl Pts',(-20.476115489232,-20.829756911557,-10.4620132410795));
#62124=CARTESIAN_POINT('Ctrl Pts',(-20.5369274194047,-20.7694302518553,
-10.4662668189649));
#62125=CARTESIAN_POINT('Ctrl Pts',(-20.5965603916463,-20.7102731421696,
-10.4704379329429));
#62126=CARTESIAN_POINT('Ctrl Pts',(-20.6533230631004,-20.6481339874866,
-10.4746090469208));
#62127=CARTESIAN_POINT('Ctrl Pts',(-20.7069098223475,-20.5833267094254,
-10.4787801608988));
#62128=CARTESIAN_POINT('Ctrl Pts',(-20.7604786000401,-20.5185411780722,
-10.4829498752192));
#62129=CARTESIAN_POINT('Ctrl Pts',(-20.8108732891326,-20.4510896556873,
-10.4871195895395));
#62130=CARTESIAN_POINT('Ctrl Pts',(-20.8578275173592,-20.3813203547519,
-10.4912893038599));
#62131=CARTESIAN_POINT('Ctrl Pts',(-20.9047800747528,-20.3115535365075,
-10.4954588698039));
#62132=CARTESIAN_POINT('Ctrl Pts',(-20.948292158553,-20.2394694858254,-10.499628435748));
#62133=CARTESIAN_POINT('Ctrl Pts',(-20.9881406062299,-20.1654455601079,
-10.503798001692));
#62134=CARTESIAN_POINT('Ctrl Pts',(-21.0293900761687,-20.0888190444805,
-10.508114164431));
#62135=CARTESIAN_POINT('Ctrl Pts',(-21.0667132396993,-20.0101141681398,
-10.5124303271699));
#62136=CARTESIAN_POINT('Ctrl Pts',(-21.0999152164605,-19.9297756330163,
-10.5167464899088));
#62137=CARTESIAN_POINT('Ctrl Pts',(-21.132035642321,-19.8520541172245,-10.5209220541005));
#62138=CARTESIAN_POINT('Ctrl Pts',(-21.160299139743,-19.7728042005822,-10.5250976182921));
#62139=CARTESIAN_POINT('Ctrl Pts',(-21.1845795982613,-19.6924455635532,
-10.5292731824838));
#62140=CARTESIAN_POINT('Ctrl Pts',(-21.210086405018,-19.6080282028024,-10.5336596444964));
#62141=CARTESIAN_POINT('Ctrl Pts',(-21.231197092147,-19.522387742153,-10.5380461065089));
#62142=CARTESIAN_POINT('Ctrl Pts',(-21.2478262226603,-19.4360224398369,
-10.5424325685214));
#62143=CARTESIAN_POINT('Ctrl Pts',(-21.2644553531735,-19.3496571375209,
-10.546819030534));
#62144=CARTESIAN_POINT('Ctrl Pts',(-21.2766029222518,-19.2625675787001,
-10.5512054925465));
#62145=CARTESIAN_POINT('Ctrl Pts',(-21.2842464642989,-19.1752553948527,
-10.555591954559));
#62146=CARTESIAN_POINT('Ctrl Pts',(-21.2907042434478,-19.1014881810632,
-10.5592979331155));
#62147=CARTESIAN_POINT('Ctrl Pts',(-21.293961988618,-19.0274367677245,-10.563003911672));
#62148=CARTESIAN_POINT('Ctrl Pts',(-21.2939996693303,-18.9533011644427,
-10.5667098902285));
#62149=CARTESIAN_POINT('Origin',(-18.734,-18.952,1.76670989022851));
#62150=CARTESIAN_POINT('',(-17.1744641548915,-16.9218650419685,-9.25004024527531));
#62151=CARTESIAN_POINT('',(-17.1750494511462,-16.9226083978001,-9.31680761352202));
#62152=CARTESIAN_POINT('',(-17.1744641548914,-16.9218650419685,1.76670989022851));
#62153=CARTESIAN_POINT('',(-21.2939992159918,-18.9540035272626,-9.8332901097715));
#62154=CARTESIAN_POINT('Ctrl Pts',(-17.1750494511459,-16.9226083978003,
-9.31680761352203));
#62155=CARTESIAN_POINT('Ctrl Pts',(-16.6852502582289,-17.3064745807427,
-9.34773678852736));
#62156=CARTESIAN_POINT('Ctrl Pts',(-15.8397231142329,-18.6405173911589,
-9.42105789909317));
#62157=CARTESIAN_POINT('Ctrl Pts',(-16.6528319614933,-21.1501880163351,
-9.53677094521944));
#62158=CARTESIAN_POINT('Ctrl Pts',(-19.4558314641724,-21.8917704497106,
-9.66394675190088));
#62159=CARTESIAN_POINT('Ctrl Pts',(-21.1196059552395,-20.3720005573578,
-9.76278617060466));
#62160=CARTESIAN_POINT('Ctrl Pts',(-21.2937096219977,-19.2372014343179,
-9.81923365374796));
#62161=CARTESIAN_POINT('Ctrl Pts',(-21.2916488755515,-18.9540199903513,
-9.83328920133079));
#62162=CARTESIAN_POINT('Ctrl Pts',(-21.2939992159918,-18.9540035272626,
-9.8332901097715));
#62163=CARTESIAN_POINT('Ctrl Pts',(-21.2940649620946,-18.8699966984849,
-9.83745593779552));
#62164=CARTESIAN_POINT('Ctrl Pts',(-21.2899913508454,-18.7859395799201,
-9.84162176581954));
#62165=CARTESIAN_POINT('Ctrl Pts',(-21.281790209728,-18.7022700514273,-9.84578759384357));
#62166=CARTESIAN_POINT('Ctrl Pts',(-21.2735905258927,-18.6186153903907,
-9.84995268163077));
#62167=CARTESIAN_POINT('Ctrl Pts',(-21.2612648140692,-18.5353486407622,
-9.85411776941798));
#62168=CARTESIAN_POINT('Ctrl Pts',(-21.244876840873,-18.4529033260305,-9.85828285720518));
#62169=CARTESIAN_POINT('Ctrl Pts',(-21.2284868533626,-18.3704478776001,
-9.86244845694076));
#62170=CARTESIAN_POINT('Ctrl Pts',(-21.2080337038202,-18.2888145159798,
-9.86661405667634));
#62171=CARTESIAN_POINT('Ctrl Pts',(-21.183632148948,-18.2084259721853,-9.87077965641192));
#62172=CARTESIAN_POINT('Ctrl Pts',(-21.1592030081949,-18.1279465493957,
-9.87494996534485));
#62173=CARTESIAN_POINT('Ctrl Pts',(-21.1308166833998,-18.0487151959126,
-9.87912027427778));
#62174=CARTESIAN_POINT('Ctrl Pts',(-21.0986375209737,-17.9711384427947,
-9.88329058321071));
#62175=CARTESIAN_POINT('Ctrl Pts',(-21.0664396371008,-17.8935165564616,
-9.88746331837886));
#62176=CARTESIAN_POINT('Ctrl Pts',(-21.0304447198543,-17.8175516031279,
-9.89163605354701));
#62177=CARTESIAN_POINT('Ctrl Pts',(-20.9908638255707,-17.7436268486802,
-9.89580878871516));
#62178=CARTESIAN_POINT('Ctrl Pts',(-20.951210438291,-17.6695666999462,-9.89998916630977));
#62179=CARTESIAN_POINT('Ctrl Pts',(-20.9079581930336,-17.5975546086432,
-9.90416954390439));
#62180=CARTESIAN_POINT('Ctrl Pts',(-20.8613622504217,-17.5279459787351,
-9.90834992149901));
#62181=CARTESIAN_POINT('Ctrl Pts',(-20.8243993123259,-17.4727278774585,
-9.91166606942059));
#62182=CARTESIAN_POINT('Ctrl Pts',(-20.7853331875372,-17.4190216712153,
-9.91498221734217));
#62183=CARTESIAN_POINT('Ctrl Pts',(-20.7443085775785,-17.3669891410737,
-9.91829836526374));
#62184=CARTESIAN_POINT('Ctrl Pts',(-20.6925397790042,-17.3013294900759,
-9.92248299965679));
#62185=CARTESIAN_POINT('Ctrl Pts',(-20.6374544461771,-17.2380865845811,
-9.92666763404984));
#62186=CARTESIAN_POINT('Ctrl Pts',(-20.5793066365797,-17.1776146368404,
-9.93085226844289));
#62187=CARTESIAN_POINT('Ctrl Pts',(-20.521241593192,-17.1172287634325,-9.93503094652683));
#62188=CARTESIAN_POINT('Ctrl Pts',(-20.4601230476225,-17.0596063422906,
-9.93920962461077));
#62189=CARTESIAN_POINT('Ctrl Pts',(-20.3962460420503,-17.0050695709173,
-9.94338830269471));
#62190=CARTESIAN_POINT('Ctrl Pts',(-20.3312240870607,-16.9495552671121,
-9.94764188058015));
#62191=CARTESIAN_POINT('Ctrl Pts',(-20.2633441071061,-16.897238700291,-9.95189545846559));
#62192=CARTESIAN_POINT('Ctrl Pts',(-20.1929575410585,-16.8484214078413,
-9.95614903635102));
#62193=CARTESIAN_POINT('Ctrl Pts',(-20.1239355559418,-16.8005505338648,
-9.96032015032898));
#62194=CARTESIAN_POINT('Ctrl Pts',(-20.0525037029721,-16.7560447387742,
-9.96449126430693));
#62195=CARTESIAN_POINT('Ctrl Pts',(-19.9790262804939,-16.7151473984905,
-9.96866237828488));
#62196=CARTESIAN_POINT('Ctrl Pts',(-19.9055735140744,-16.6742637817044,
-9.97283209260525));
#62197=CARTESIAN_POINT('Ctrl Pts',(-19.8300769429975,-16.6369864384996,
-9.97700180692563));
#62198=CARTESIAN_POINT('Ctrl Pts',(-19.7529274425307,-16.6035139202333,
-9.981171521246));
#62199=CARTESIAN_POINT('Ctrl Pts',(-19.6757806873741,-16.5700425930628,
-9.98534108719004));
#62200=CARTESIAN_POINT('Ctrl Pts',(-19.5969815421365,-16.5403760039566,
-9.98951065313409));
#62201=CARTESIAN_POINT('Ctrl Pts',(-19.5169416763859,-16.5146649119627,
-9.99368021907813));
#62202=CARTESIAN_POINT('Ctrl Pts',(-19.4340877076954,-16.4880498496923,
-9.99799638181705));
#62203=CARTESIAN_POINT('Ctrl Pts',(-19.3499046498555,-16.4656737716516,
-10.002312544556));
#62204=CARTESIAN_POINT('Ctrl Pts',(-19.264865245119,-16.4476473707713,-10.0066287072949));
#62205=CARTESIAN_POINT('Ctrl Pts',(-19.1825959900472,-16.4302081780036,
-10.0108042714866));
#62206=CARTESIAN_POINT('Ctrl Pts',(-19.0995257948678,-16.4168396609884,
-10.0149798356783));
#62207=CARTESIAN_POINT('Ctrl Pts',(-19.0160902825553,-16.4075894449818,
-10.0191553998699));
#62208=CARTESIAN_POINT('Ctrl Pts',(-18.928440640865,-16.397872022555,-10.0235418618825));
#62209=CARTESIAN_POINT('Ctrl Pts',(-18.8403883907189,-16.3926998996315,
-10.027928323895));
#62210=CARTESIAN_POINT('Ctrl Pts',(-18.7524390182802,-16.3920664066025,
-10.0323147859076));
#62211=CARTESIAN_POINT('Ctrl Pts',(-18.6644896458415,-16.3914329135735,
-10.0367012479201));
#62212=CARTESIAN_POINT('Ctrl Pts',(-18.5766437273768,-16.395337948682,-10.0410877099327));
#62213=CARTESIAN_POINT('Ctrl Pts',(-18.4893986055749,-16.403712308658,-10.0454741719452));
#62214=CARTESIAN_POINT('Ctrl Pts',(-18.4061740830955,-16.4117007450963,
-10.0496584884872));
#62215=CARTESIAN_POINT('Ctrl Pts',(-18.3231864480459,-16.4237853774939,
-10.0538428050293));
#62216=CARTESIAN_POINT('Ctrl Pts',(-18.2408709541789,-16.4399443190551,
-10.0580271215713));
#62217=CARTESIAN_POINT('Ctrl Pts',(-18.1586671962098,-16.4560813263029,
-10.062205758279));
#62218=CARTESIAN_POINT('Ctrl Pts',(-18.0771342151715,-16.4762815730405,
-10.0663843949868));
#62219=CARTESIAN_POINT('Ctrl Pts',(-17.9967026166349,-16.5004713812637,
-10.0705630316945));
#62220=CARTESIAN_POINT('Ctrl Pts',(-17.9163646373239,-16.5246330334991,
-10.074736804633));
#62221=CARTESIAN_POINT('Ctrl Pts',(-17.8371259305098,-16.5527748851385,
-10.0789105775716));
#62222=CARTESIAN_POINT('Ctrl Pts',(-17.7594058894995,-16.5847724402209,
-10.0830843505101));
#62223=CARTESIAN_POINT('Ctrl Pts',(-17.6817391960101,-16.6167480319819,
-10.0872552585448));
#62224=CARTESIAN_POINT('Ctrl Pts',(-17.6055895218756,-16.6525738957107,
-10.0914261665796));
#62225=CARTESIAN_POINT('Ctrl Pts',(-17.5313590153092,-16.6920764035167,
-10.0955970746143));
#62226=CARTESIAN_POINT('Ctrl Pts',(-17.4571459112411,-16.7315696504089,
-10.0997670048271));
#62227=CARTESIAN_POINT('Ctrl Pts',(-17.3848514901433,-16.7747376197236,
-10.1039369350399));
#62228=CARTESIAN_POINT('Ctrl Pts',(-17.3148548334046,-16.821359956227,-10.1081068652527));
#62229=CARTESIAN_POINT('Ctrl Pts',(-17.2669439265524,-16.8532717435255,
-10.1109610749723));
#62230=CARTESIAN_POINT('Ctrl Pts',(-17.2201090559903,-16.8868009398858,
-10.1138152846919));
#62231=CARTESIAN_POINT('Ctrl Pts',(-17.1744641548914,-16.9218650419685,
-10.1166694944115));
#62232=CARTESIAN_POINT('',(-21.2939989766127,-18.9497109517324,-9.7667098901893));
#62233=CARTESIAN_POINT('Ctrl Pts',(-21.293998976612,-18.9497109509451,-9.76670989022851));
#62234=CARTESIAN_POINT('Ctrl Pts',(-21.2938920610985,-18.8301400729742,
-9.77266511192846));
#62235=CARTESIAN_POINT('Ctrl Pts',(-21.2854044483395,-18.7109297707717,
-9.77862033362841));
#62236=CARTESIAN_POINT('Ctrl Pts',(-21.2687069780221,-18.5930285031284,
-9.78457555532836));
#62237=CARTESIAN_POINT('Ctrl Pts',(-21.2612660069352,-18.5404876147807,
-9.78722940837572));
#62238=CARTESIAN_POINT('Ctrl Pts',(-21.2521952261608,-18.4882062515499,
-9.78988326142308));
#62239=CARTESIAN_POINT('Ctrl Pts',(-21.2415125421986,-18.4362666864387,
-9.79253711447044));
#62240=CARTESIAN_POINT('Ctrl Pts',(-21.2246679295087,-18.3543676186888,
-9.79672174886349));
#62241=CARTESIAN_POINT('Ctrl Pts',(-21.2037753333229,-18.2731422629634,
-9.80090638325654));
#62242=CARTESIAN_POINT('Ctrl Pts',(-21.1789030820534,-18.1930211337819,
-9.80509101764958));
#62243=CARTESIAN_POINT('Ctrl Pts',(-21.1540662333551,-18.1130140471107,
-9.80926969573353));
#62244=CARTESIAN_POINT('Ctrl Pts',(-21.125261116367,-18.0341085006255,-9.81344837381748));
#62245=CARTESIAN_POINT('Ctrl Pts',(-21.0926070466711,-17.9567247619913,
-9.81762705190143));
#62246=CARTESIAN_POINT('Ctrl Pts',(-21.059367676244,-17.8779539754568,-9.82188062978687));
#62247=CARTESIAN_POINT('Ctrl Pts',(-21.022140108072,-17.8007605624569,-9.8261342076723));
#62248=CARTESIAN_POINT('Ctrl Pts',(-20.9811033321017,-17.7255716022296,
-9.83038778555774));
#62249=CARTESIAN_POINT('Ctrl Pts',(-20.9408621341102,-17.6518403267155,
-9.83455889953569));
#62250=CARTESIAN_POINT('Ctrl Pts',(-20.8969583386824,-17.5800368994828,
-9.83873001351364));
#62251=CARTESIAN_POINT('Ctrl Pts',(-20.8496085018329,-17.5105421730164,
-9.84290112749159));
#62252=CARTESIAN_POINT('Ctrl Pts',(-20.8022745536785,-17.4410707661766,
-9.84707084181197));
#62253=CARTESIAN_POINT('Ctrl Pts',(-20.7514971194517,-17.3739069013821,
-9.85124055613235));
#62254=CARTESIAN_POINT('Ctrl Pts',(-20.69753660511,-17.3094032751789,-9.85541027045272));
#62255=CARTESIAN_POINT('Ctrl Pts',(-20.643578010915,-17.2449019442916,-9.85957983639677));
#62256=CARTESIAN_POINT('Ctrl Pts',(-20.5864368576392,-17.1830610160831,
-9.86374940234081));
#62257=CARTESIAN_POINT('Ctrl Pts',(-20.5264135623406,-17.1241997862082,
-9.86791896828485));
#62258=CARTESIAN_POINT('Ctrl Pts',(-20.4642799220261,-17.063269068104,-9.87223513102377));
#62259=CARTESIAN_POINT('Ctrl Pts',(-20.3990580731256,-17.0055318485508,
-9.87655129376269));
#62260=CARTESIAN_POINT('Ctrl Pts',(-20.3311209857106,-16.9512989836053,
-9.88086745650161));
#62261=CARTESIAN_POINT('Ctrl Pts',(-20.2653969417724,-16.8988327485311,
-9.88504302069329));
#62262=CARTESIAN_POINT('Ctrl Pts',(-20.1971322502977,-16.84964630251,-9.88921858488496));
#62263=CARTESIAN_POINT('Ctrl Pts',(-20.1266949702185,-16.8039774861682,
-9.89339414907664));
#62264=CARTESIAN_POINT('Ctrl Pts',(-20.0527000705712,-16.7560020464804,
-9.89778061108918));
#62265=CARTESIAN_POINT('Ctrl Pts',(-19.9763078452048,-16.7119092180967,
-9.90216707310172));
#62266=CARTESIAN_POINT('Ctrl Pts',(-19.8979731420051,-16.6719196231951,
-9.90655353511426));
#62267=CARTESIAN_POINT('Ctrl Pts',(-19.8196384388055,-16.6319300282936,
-9.9109399971268));
#62268=CARTESIAN_POINT('Ctrl Pts',(-19.7393618185146,-16.5960438342244,
-9.91532645913934));
#62269=CARTESIAN_POINT('Ctrl Pts',(-19.6576188802165,-16.5644221134992,
-9.91971292115188));
#62270=CARTESIAN_POINT('Ctrl Pts',(-19.5796370556816,-16.5342553550192,
-9.92389755554493));
#62271=CARTESIAN_POINT('Ctrl Pts',(-19.5000306196518,-16.5078569775931,
-9.92808218993798));
#62272=CARTESIAN_POINT('Ctrl Pts',(-19.4191985515812,-16.4854025571831,
-9.93226682433103));
#62273=CARTESIAN_POINT('Ctrl Pts',(-19.3384815379545,-16.4629800978612,
-9.93644550241497));
#62274=CARTESIAN_POINT('Ctrl Pts',(-19.2565427969406,-16.4444905669892,
-9.94062418049891));
#62275=CARTESIAN_POINT('Ctrl Pts',(-19.1738002903985,-16.4300611219609,
-9.94480285858285));
#62276=CARTESIAN_POINT('Ctrl Pts',(-19.0895746838926,-16.4153730395006,
-9.94905643646829));
#62277=CARTESIAN_POINT('Ctrl Pts',(-19.0045166631073,-16.404892202575,-9.95331001435372));
#62278=CARTESIAN_POINT('Ctrl Pts',(-18.9190822179583,-16.3986992788558,
-9.95756359223916));
#62279=CARTESIAN_POINT('Ctrl Pts',(-18.8353040862402,-16.3926264170474,
-9.96173470621711));
#62280=CARTESIAN_POINT('Ctrl Pts',(-18.7511644753125,-16.3906767277746,
-9.96590582019506));
#62281=CARTESIAN_POINT('Ctrl Pts',(-18.6671008395072,-16.3928742699263,
-9.97007693417301));
#62282=CARTESIAN_POINT('Ctrl Pts',(-18.5830654120667,-16.3950710746715,
-9.97424664849338));
#62283=CARTESIAN_POINT('Ctrl Pts',(-18.4991063686099,-16.4014123350032,
-9.97841636281376));
#62284=CARTESIAN_POINT('Ctrl Pts',(-18.4156612239222,-16.4118699986723,
-9.98258607713413));
#62285=CARTESIAN_POINT('Ctrl Pts',(-18.3322190485708,-16.4223272902128,
-9.98675564307817));
#62286=CARTESIAN_POINT('Ctrl Pts',(-18.249291191986,-16.4369006358009,-9.99092520902222));
#62287=CARTESIAN_POINT('Ctrl Pts',(-18.1673087413395,-16.4555102609148,
-9.99509477496626));
#62288=CARTESIAN_POINT('Ctrl Pts',(-18.0824438888645,-16.4747741774902,
-9.99941093770518));
#62289=CARTESIAN_POINT('Ctrl Pts',(-17.9985926745536,-16.498363368963,-10.0037271004441));
#62290=CARTESIAN_POINT('Ctrl Pts',(-17.9162183607824,-16.5261324870145,
-10.008043263183));
#62291=CARTESIAN_POINT('Ctrl Pts',(-17.836527381618,-16.5529970289662,-10.0122188273747));
#62292=CARTESIAN_POINT('Ctrl Pts',(-17.7582189816851,-16.5837731410384,
-10.0163943915664));
#62293=CARTESIAN_POINT('Ctrl Pts',(-17.6816923706303,-16.6182800825355,
-10.0205699557581));
#62294=CARTESIAN_POINT('Ctrl Pts',(-17.6013005823759,-16.6545298876153,
-10.0249564177706));
#62295=CARTESIAN_POINT('Ctrl Pts',(-17.5228758288488,-16.6948970480992,
-10.0293428797832));
#62296=CARTESIAN_POINT('Ctrl Pts',(-17.4468498189204,-16.7391185274971,
-10.0337293417957));
#62297=CARTESIAN_POINT('Ctrl Pts',(-17.3708238089919,-16.7833400068949,
-10.0381158038082));
#62298=CARTESIAN_POINT('Ctrl Pts',(-17.2971969868961,-16.8314154242948,
-10.0425022658208));
#62299=CARTESIAN_POINT('Ctrl Pts',(-17.2263622218887,-16.8830320616279,
-10.0468887278333));
#62300=CARTESIAN_POINT('Ctrl Pts',(-17.2089081327501,-16.8957506947588,
-10.0479695770316));
#62301=CARTESIAN_POINT('Ctrl Pts',(-17.1916066348401,-16.9086963056497,
-10.0490504262299));
#62302=CARTESIAN_POINT('Ctrl Pts',(-17.1744641548914,-16.9218650419685,
-10.0501312754282));
#62303=CARTESIAN_POINT('Ctrl Pts',(-17.1744641548915,-16.9218650419685,
-9.25004024527531));
#62304=CARTESIAN_POINT('Ctrl Pts',(-17.1077983713942,-16.9730772427116,
-9.25421688536645));
#62305=CARTESIAN_POINT('Ctrl Pts',(-17.0437156465026,-17.0275321795368,
-9.25839352545759));
#62306=CARTESIAN_POINT('Ctrl Pts',(-16.9825323038481,-17.0849271815657,
-9.26257016554873));
#62307=CARTESIAN_POINT('Ctrl Pts',(-16.9212437929918,-17.1424208400081,
-9.26675398487704));
#62308=CARTESIAN_POINT('Ctrl Pts',(-16.8628649371421,-17.2028643252882,
-9.27093780420536));
#62309=CARTESIAN_POINT('Ctrl Pts',(-16.8076737517062,-17.2659195792803,
-9.27512162353367));
#62310=CARTESIAN_POINT('Ctrl Pts',(-16.7693642429451,-17.3096877242506,
-9.27802571160402));
#62311=CARTESIAN_POINT('Ctrl Pts',(-16.7325897413083,-17.3547135268183,
-9.28092979967436));
#62312=CARTESIAN_POINT('Ctrl Pts',(-16.6974308899392,-17.4008758076974,
-9.28383388774471));
#62313=CARTESIAN_POINT('Ctrl Pts',(-16.6467688800086,-17.4673931665203,
-9.28801852213775));
#62314=CARTESIAN_POINT('Ctrl Pts',(-16.5992748500801,-17.5365189656784,
-9.2922031565308));
#62315=CARTESIAN_POINT('Ctrl Pts',(-16.5552283987657,-17.6079187860643,
-9.29638779092385));
#62316=CARTESIAN_POINT('Ctrl Pts',(-16.5112446421229,-17.6792169776433,
-9.3005664690078));
#62317=CARTESIAN_POINT('Ctrl Pts',(-16.4706989563139,-17.7527823729939,
-9.30474514709174));
#62318=CARTESIAN_POINT('Ctrl Pts',(-16.4338297096935,-17.8282488551323,
-9.30892382517568));
#62319=CARTESIAN_POINT('Ctrl Pts',(-16.3962996083249,-17.9050680197263,
-9.31317740306112));
#62320=CARTESIAN_POINT('Ctrl Pts',(-16.3625793350038,-17.9838567118701,
-9.31743098094656));
#62321=CARTESIAN_POINT('Ctrl Pts',(-16.3328731767861,-18.0641993586154,
-9.32168455883199));
#62322=CARTESIAN_POINT('Ctrl Pts',(-16.3037429304123,-18.1429844063778,
-9.32585567280994));
#62323=CARTESIAN_POINT('Ctrl Pts',(-16.2784727120491,-18.223263242189,-9.33002678678789));
#62324=CARTESIAN_POINT('Ctrl Pts',(-16.2572072783656,-18.3046223559168,
-9.33419790076585));
#62325=CARTESIAN_POINT('Ctrl Pts',(-16.2359489805037,-18.3859541688082,
-9.33836761508622));
#62326=CARTESIAN_POINT('Ctrl Pts',(-16.2186929146628,-18.4683650949799,
-9.34253732940659));
#62327=CARTESIAN_POINT('Ctrl Pts',(-16.2055337985359,-18.5514270752364,
-9.34670704372697));
#62328=CARTESIAN_POINT('Ctrl Pts',(-16.1923751506668,-18.6344860997912,
-9.35087660967101));
#62329=CARTESIAN_POINT('Ctrl Pts',(-16.183313233791,-18.7181956778687,-9.35504617561505));
#62330=CARTESIAN_POINT('Ctrl Pts',(-16.1783912959603,-18.8021195415123,
-9.3592157415591));
#62331=CARTESIAN_POINT('Ctrl Pts',(-16.1732963088673,-18.8889940646704,
-9.36353190429802));
#62332=CARTESIAN_POINT('Ctrl Pts',(-16.1726378716504,-18.9760976958013,
-9.36784806703694));
#62333=CARTESIAN_POINT('Ctrl Pts',(-16.1764051921424,-19.0629450261169,
-9.37216422977586));
#62334=CARTESIAN_POINT('Ctrl Pts',(-16.1800497925657,-19.1469633137821,
-9.37633979396754));
#62335=CARTESIAN_POINT('Ctrl Pts',(-16.1878361499306,-19.2307412775514,
-9.38051535815922));
#62336=CARTESIAN_POINT('Ctrl Pts',(-16.1997016639331,-19.3138451931539,
-9.3846909223509));
#62337=CARTESIAN_POINT('Ctrl Pts',(-16.2121664768403,-19.4011464899727,
-9.38907738436344));
#62338=CARTESIAN_POINT('Ctrl Pts',(-16.2291332400404,-19.487703283801,-9.39346384637598));
#62339=CARTESIAN_POINT('Ctrl Pts',(-16.2504693406595,-19.5730277482654,
-9.39785030838852));
#62340=CARTESIAN_POINT('Ctrl Pts',(-16.2718054412786,-19.6583522127299,
-9.40223677040106));
#62341=CARTESIAN_POINT('Ctrl Pts',(-16.2975106369606,-19.7424438151944,
-9.4066232324136));
#62342=CARTESIAN_POINT('Ctrl Pts',(-16.3273937923111,-19.8248382216157,
-9.41100969442614));
#62343=CARTESIAN_POINT('Ctrl Pts',(-16.3559019793865,-19.9034415392598,
-9.41519432881919));
#62344=CARTESIAN_POINT('Ctrl Pts',(-16.3883182194788,-19.9807929863463,
-9.41937896321224));
#62345=CARTESIAN_POINT('Ctrl Pts',(-16.4245126604672,-20.0564764499698,
-9.42356359760528));
#62346=CARTESIAN_POINT('Ctrl Pts',(-16.460655583149,-20.1320521875506,-9.42774227568923));
#62347=CARTESIAN_POINT('Ctrl Pts',(-16.5005658279439,-20.2059642460473,
-9.43192095377317));
#62348=CARTESIAN_POINT('Ctrl Pts',(-16.5440645726776,-20.2778140232167,
-9.43609963185712));
#62349=CARTESIAN_POINT('Ctrl Pts',(-16.5883430011486,-20.3509516560044,
-9.44035320974255));
#62350=CARTESIAN_POINT('Ctrl Pts',(-16.6363396782675,-20.4219518942302,
-9.44460678762799));
#62351=CARTESIAN_POINT('Ctrl Pts',(-16.6878157496594,-20.4904180230543,
-9.44886036551343));
#62352=CARTESIAN_POINT('Ctrl Pts',(-16.7382938569602,-20.5575568023704,
-9.45303147949138));
#62353=CARTESIAN_POINT('Ctrl Pts',(-16.7921173635638,-20.6222584681312,
-9.45720259346933));
#62354=CARTESIAN_POINT('Ctrl Pts',(-16.8490169269279,-20.6841774776944,
-9.46137370744728));
#62355=CARTESIAN_POINT('Ctrl Pts',(-16.905897397094,-20.746075709736,-9.46554342176766));
#62356=CARTESIAN_POINT('Ctrl Pts',(-16.9658515630401,-20.8051928015664,
-9.46971313608803));
#62357=CARTESIAN_POINT('Ctrl Pts',(-17.0285707636154,-20.8612174102717,
-9.4738828504084));
#62358=CARTESIAN_POINT('Ctrl Pts',(-17.0912877323723,-20.9172400253809,
-9.47805241635245));
#62359=CARTESIAN_POINT('Ctrl Pts',(-17.1567691964755,-20.9701700703297,
-9.48222198229649));
#62360=CARTESIAN_POINT('Ctrl Pts',(-17.2246717329647,-21.0197350367801,
-9.48639154824053));
#62361=CARTESIAN_POINT('Ctrl Pts',(-17.2949616388699,-21.071042646306,-9.49070771097946));
#62362=CARTESIAN_POINT('Ctrl Pts',(-17.3678456086252,-21.1187438312856,
-9.49502387371838));
#62363=CARTESIAN_POINT('Ctrl Pts',(-17.4429096486621,-21.1625849236531,
-9.4993400364573));
#62364=CARTESIAN_POINT('Ctrl Pts',(-17.5155284854901,-21.2049978970479,
-9.50351560064898));
#62365=CARTESIAN_POINT('Ctrl Pts',(-17.5901871024315,-21.2437982255354,
-9.50769116484066));
#62366=CARTESIAN_POINT('Ctrl Pts',(-17.6664869216557,-21.2788037793428,
-9.51186672903234));
#62367=CARTESIAN_POINT('Ctrl Pts',(-17.7466404633634,-21.3155773804553,
-9.51625319104488));
#62368=CARTESIAN_POINT('Ctrl Pts',(-17.8286048161834,-21.3481625684723,
-9.52063965305742));
#62369=CARTESIAN_POINT('Ctrl Pts',(-17.9118980145027,-21.3764067986709,
-9.52502611506996));
#62370=CARTESIAN_POINT('Ctrl Pts',(-17.9951912128221,-21.4046510288695,
-9.5294125770825));
#62371=CARTESIAN_POINT('Ctrl Pts',(-18.0798126775953,-21.428554216727,-9.53379903909504));
#62372=CARTESIAN_POINT('Ctrl Pts',(-18.1652685194105,-21.4480257416514,
-9.53818550110758));
#62373=CARTESIAN_POINT('Ctrl Pts',(-18.2467924112678,-21.4666013528503,
-9.54237013550063));
#62374=CARTESIAN_POINT('Ctrl Pts',(-18.3293790330749,-21.4812132961356,
-9.54655476989367));
#62375=CARTESIAN_POINT('Ctrl Pts',(-18.4126082132397,-21.4917455225678,
-9.55073940428672));
#62376=CARTESIAN_POINT('Ctrl Pts',(-18.4957189269682,-21.5022627576792,
-9.55491808237066));
#62377=CARTESIAN_POINT('Ctrl Pts',(-18.5794699298769,-21.508711753151,-9.5590967604546));
#62378=CARTESIAN_POINT('Ctrl Pts',(-18.663429267508,-21.5110271142986,-9.56327543853855));
#62379=CARTESIAN_POINT('Ctrl Pts',(-18.7488935159256,-21.5133839766308,
-9.56752901642398));
#62380=CARTESIAN_POINT('Ctrl Pts',(-18.8345731712377,-21.5114574491383,
-9.57178259430942));
#62381=CARTESIAN_POINT('Ctrl Pts',(-18.9200053717025,-21.5052336363321,
-9.57603617219485));
#62382=CARTESIAN_POINT('Ctrl Pts',(-19.0037813022541,-21.499130484282,-9.58020728617281));
#62383=CARTESIAN_POINT('Ctrl Pts',(-19.0873188071793,-21.4888952174951,
-9.58437840015076));
#62384=CARTESIAN_POINT('Ctrl Pts',(-19.1701815497897,-21.4745672747467,
-9.58854951412871));
#62385=CARTESIAN_POINT('Ctrl Pts',(-19.2530164870065,-21.4602441398779,
-9.59271922844908));
#62386=CARTESIAN_POINT('Ctrl Pts',(-19.3351766586593,-21.4418311348332,
-9.59688894276946));
#62387=CARTESIAN_POINT('Ctrl Pts',(-19.4162332022015,-21.4194192707795,
-9.60105865708983));
#62388=CARTESIAN_POINT('Ctrl Pts',(-19.497286861404,-21.3970082042361,-9.60522822303387));
#62389=CARTESIAN_POINT('Ctrl Pts',(-19.5772365274095,-21.3705986850247,
-9.60939778897791));
#62390=CARTESIAN_POINT('Ctrl Pts',(-19.6556671754964,-21.3403319739124,
-9.61356735492195));
#62391=CARTESIAN_POINT('Ctrl Pts',(-19.7368553484154,-21.3090011225755,
-9.61788351766088));
#62392=CARTESIAN_POINT('Ctrl Pts',(-19.8164152065818,-21.2735369848544,
-9.6221996803998));
#62393=CARTESIAN_POINT('Ctrl Pts',(-19.8939093684295,-21.2341503581117,
-9.62651584313872));
#62394=CARTESIAN_POINT('Ctrl Pts',(-19.9688791661059,-21.1960467465925,
-9.63069140733039));
#62395=CARTESIAN_POINT('Ctrl Pts',(-20.0419153954164,-21.1542725466308,
-9.63486697152208));
#62396=CARTESIAN_POINT('Ctrl Pts',(-20.112649171425,-21.1090643157146,-9.63904253571376));
#62397=CARTESIAN_POINT('Ctrl Pts',(-20.1869555423062,-21.0615727245271,
-9.6434289977263));
#62398=CARTESIAN_POINT('Ctrl Pts',(-20.2587202783153,-21.0102914191921,
-9.64781545973884));
#62399=CARTESIAN_POINT('Ctrl Pts',(-20.3275542346358,-20.9555430869523,
-9.65220192175138));
#62400=CARTESIAN_POINT('Ctrl Pts',(-20.3963881909563,-20.9007947547124,
-9.65658838376392));
#62401=CARTESIAN_POINT('Ctrl Pts',(-20.4622909830917,-20.8425798367028,
-9.66097484577646));
#62402=CARTESIAN_POINT('Ctrl Pts',(-20.5249190804939,-20.7812645645513,
-9.665361307789));
#62403=CARTESIAN_POINT('Ctrl Pts',(-20.5852113014986,-20.722236203594,-9.66958416538901));
#62404=CARTESIAN_POINT('Ctrl Pts',(-20.6427127908697,-20.6600954577448,
-9.67380702298902));
#62405=CARTESIAN_POINT('Ctrl Pts',(-20.6970796830689,-20.5951427685755,
-9.67802988058904));
#62406=CARTESIAN_POINT('Ctrl Pts',(-20.7500936846377,-20.5318063918539,
-9.68214765466763));
#62407=CARTESIAN_POINT('Ctrl Pts',(-20.8001269202378,-20.465796754398,-9.68626542874623));
#62408=CARTESIAN_POINT('Ctrl Pts',(-20.8468954124061,-20.3974317611819,
-9.69038320282483));
#62409=CARTESIAN_POINT('Ctrl Pts',(-20.89361966769,-20.3291314323191,-9.69449708202704));
#62410=CARTESIAN_POINT('Ctrl Pts',(-20.9370850392269,-20.2584805564847,
-9.69861096122924));
#62411=CARTESIAN_POINT('Ctrl Pts',(-20.9770478427321,-20.1858299620349,
-9.70272484043145));
#62412=CARTESIAN_POINT('Ctrl Pts',(-21.0169856434319,-20.1132248215702,
-9.70683614577717));
#62413=CARTESIAN_POINT('Ctrl Pts',(-21.0534249974543,-20.038622860247,-9.71094745112288));
#62414=CARTESIAN_POINT('Ctrl Pts',(-21.0861664418207,-19.9624024099201,
-9.7150587564686));
#62415=CARTESIAN_POINT('Ctrl Pts',(-21.1204445396302,-19.88260470698,-9.71936301761199));
#62416=CARTESIAN_POINT('Ctrl Pts',(-21.1506688210158,-19.8010333411259,
-9.72366727875538));
#62417=CARTESIAN_POINT('Ctrl Pts',(-21.1766659614561,-19.7181481584811,
-9.72797153989877));
#62418=CARTESIAN_POINT('Ctrl Pts',(-21.2014998963995,-19.6389715567968,
-9.73208321292912));
#62419=CARTESIAN_POINT('Ctrl Pts',(-21.222476755318,-19.5585966865054,-9.73619488595946));
#62420=CARTESIAN_POINT('Ctrl Pts',(-21.2394965458156,-19.4774398718274,
-9.74030655898981));
#62421=CARTESIAN_POINT('Ctrl Pts',(-21.2565208804896,-19.3962613887936,
-9.74441932981082));
#62422=CARTESIAN_POINT('Ctrl Pts',(-21.2695859645564,-19.3143010135805,
-9.74853210063183));
#62423=CARTESIAN_POINT('Ctrl Pts',(-21.2786432445868,-19.2319834955467,
-9.75264487145285));
#62424=CARTESIAN_POINT('Ctrl Pts',(-21.2877094512626,-19.1495848472747,
-9.75676169572548));
#62425=CARTESIAN_POINT('Ctrl Pts',(-21.2927599450141,-19.066828826857,-9.76087851999811));
#62426=CARTESIAN_POINT('Ctrl Pts',(-21.2937982075177,-18.9841424452888,
-9.76499534427074));
#62427=CARTESIAN_POINT('Ctrl Pts',(-21.2939423435977,-18.9726635650768,
-9.76556685957692));
#62428=CARTESIAN_POINT('Ctrl Pts',(-21.2940092371596,-18.9611860219109,
-9.76613837488311));
#62429=CARTESIAN_POINT('Ctrl Pts',(-21.2939989766127,-18.9497109517324,
-9.7667098901893));
#62430=CARTESIAN_POINT('Origin',(-18.734,-18.952,1.76670989022851));
#62431=CARTESIAN_POINT('',(-17.1744641548914,-16.9218650419685,-8.45013430174985));
#62432=CARTESIAN_POINT('',(-17.1744641548914,-16.9218650419685,-8.51667714937936));
#62433=CARTESIAN_POINT('',(-17.1744641548914,-16.9218650419685,1.76670989022851));
#62434=CARTESIAN_POINT('',(-21.294330140624,-18.9526425111494,-9.03329016589256));
#62435=CARTESIAN_POINT('Ctrl Pts',(-17.1744641548914,-16.9218650419685,
-8.51667714937936));
#62436=CARTESIAN_POINT('Ctrl Pts',(-17.160259116072,-16.9327772560222,-8.51757293017557));
#62437=CARTESIAN_POINT('Ctrl Pts',(-17.1461740119804,-16.9438344208981,
-8.51846871097177));
#62438=CARTESIAN_POINT('Ctrl Pts',(-17.1322119090441,-16.9550335727229,
-8.51936449176797));
#62439=CARTESIAN_POINT('Ctrl Pts',(-17.0669880324056,-17.0073503405056,
-8.52354912616102));
#62440=CARTESIAN_POINT('Ctrl Pts',(-17.0042085866859,-17.0629632902854,
-8.52773376055407));
#62441=CARTESIAN_POINT('Ctrl Pts',(-16.9442256444346,-17.1216154075822,
-8.53191839494711));
#62442=CARTESIAN_POINT('Ctrl Pts',(-16.8843280804771,-17.1801840408498,
-8.53609707303105));
#62443=CARTESIAN_POINT('Ctrl Pts',(-16.8272194396166,-17.2417829302055,
-8.540275751115));
#62444=CARTESIAN_POINT('Ctrl Pts',(-16.7732194376016,-17.3061143459764,
-8.54445442919894));
#62445=CARTESIAN_POINT('Ctrl Pts',(-16.7182515243597,-17.3715988561408,
-8.54870800708437));
#62446=CARTESIAN_POINT('Ctrl Pts',(-16.6665051669308,-17.4399145156591,
-8.55296158496981));
#62447=CARTESIAN_POINT('Ctrl Pts',(-16.6182789494494,-17.5107073731345,
-8.55721516285525));
#62448=CARTESIAN_POINT('Ctrl Pts',(-16.5709876912995,-17.5801277729268,
-8.5613862768332));
#62449=CARTESIAN_POINT('Ctrl Pts',(-16.5270815724709,-17.6519297794777,
-8.56555739081115));
#62450=CARTESIAN_POINT('Ctrl Pts',(-16.4868009099953,-17.7257470693687,
-8.5697285047891));
#62451=CARTESIAN_POINT('Ctrl Pts',(-16.446533764085,-17.7995395891551,-8.57389821910947));
#62452=CARTESIAN_POINT('Ctrl Pts',(-16.409889878601,-17.8753456457563,-8.57806793342985));
#62453=CARTESIAN_POINT('Ctrl Pts',(-16.3770645250475,-17.952772715089,-8.58223764775022));
#62454=CARTESIAN_POINT('Ctrl Pts',(-16.344240339561,-18.0301970292344,-8.58640721369426));
#62455=CARTESIAN_POINT('Ctrl Pts',(-16.315234594618,-18.1092418175489,-8.59057677963831));
#62456=CARTESIAN_POINT('Ctrl Pts',(-16.2901945969736,-18.1894941625542,
-8.59474634558235));
#62457=CARTESIAN_POINT('Ctrl Pts',(-16.2642742239021,-18.2725680810079,
-8.59906250832127));
#62458=CARTESIAN_POINT('Ctrl Pts',(-16.2426038152403,-18.3569355479853,
-8.60337867106019));
#62459=CARTESIAN_POINT('Ctrl Pts',(-16.2252901016539,-18.4421229109477,
-8.60769483379911));
#62460=CARTESIAN_POINT('Ctrl Pts',(-16.2085403804665,-18.5245353045217,
-8.61187039799079));
#62461=CARTESIAN_POINT('Ctrl Pts',(-16.1958678987932,-18.6077145253799,
-8.61604596218247));
#62462=CARTESIAN_POINT('Ctrl Pts',(-16.1873166326445,-18.6912245670412,
-8.62022152637415));
#62463=CARTESIAN_POINT('Ctrl Pts',(-16.1783334623714,-18.7789525023805,
-8.62460798838669));
#62464=CARTESIAN_POINT('Ctrl Pts',(-16.1738988033979,-18.8670449731774,
-8.62899445039923));
#62465=CARTESIAN_POINT('Ctrl Pts',(-16.1740017537922,-18.9549965668354,
-8.63338091241177));
#62466=CARTESIAN_POINT('Ctrl Pts',(-16.1741047041864,-19.0429481604934,
-8.63776737442431));
#62467=CARTESIAN_POINT('Ctrl Pts',(-16.1787451573697,-19.1307583016182,
-8.64215383643685));
#62468=CARTESIAN_POINT('Ctrl Pts',(-16.1878497481281,-19.2179302444114,
-8.64654029844939));
#62469=CARTESIAN_POINT('Ctrl Pts',(-16.1965354231695,-19.3010912768969,
-8.65072493284244));
#62470=CARTESIAN_POINT('Ctrl Pts',(-16.2093157897326,-19.3839810906174,
-8.65490956723549));
#62471=CARTESIAN_POINT('Ctrl Pts',(-16.2261653095063,-19.4661645312117,
-8.65909420162853));
#62472=CARTESIAN_POINT('Ctrl Pts',(-16.2429908460741,-19.5482309938506,
-8.66327287971248));
#62473=CARTESIAN_POINT('Ctrl Pts',(-16.2638739396399,-19.629592633669,-8.66745155779642));
#62474=CARTESIAN_POINT('Ctrl Pts',(-16.2887373027363,-19.7098194648929,
-8.67163023588037));
#62475=CARTESIAN_POINT('Ctrl Pts',(-16.3140463237472,-19.7914843044086,
-8.6758838137658));
#62476=CARTESIAN_POINT('Ctrl Pts',(-16.3434796603857,-19.871972772756,-8.68013739165124));
#62477=CARTESIAN_POINT('Ctrl Pts',(-16.3769013134697,-19.9508422207522,
-8.68439096953667));
#62478=CARTESIAN_POINT('Ctrl Pts',(-16.4096750225917,-20.0281826305979,
-8.68856208351462));
#62479=CARTESIAN_POINT('Ctrl Pts',(-16.4462835978106,-20.103965792552,-8.69273319749258));
#62480=CARTESIAN_POINT('Ctrl Pts',(-16.4865490981546,-20.1777913541033,
-8.69690431147053));
#62481=CARTESIAN_POINT('Ctrl Pts',(-16.5268010870211,-20.2515921427744,
-8.7010740257909));
#62482=CARTESIAN_POINT('Ctrl Pts',(-16.5707073438479,-20.3234362321085,
-8.70524374011128));
#62483=CARTESIAN_POINT('Ctrl Pts',(-16.618043514761,-20.3929469638315,-8.70941345443165));
#62484=CARTESIAN_POINT('Ctrl Pts',(-16.66537800125,-20.4624552220643,-8.71358302037569));
#62485=CARTESIAN_POINT('Ctrl Pts',(-16.7161418995133,-20.5296299080143,
-8.71775258631974));
#62486=CARTESIAN_POINT('Ctrl Pts',(-16.77006774565,-20.594123655613,-8.72192215226378));
#62487=CARTESIAN_POINT('Ctrl Pts',(-16.8258895580122,-20.6608849238157,
-8.7262383150027));
#62488=CARTESIAN_POINT('Ctrl Pts',(-16.8850994651022,-20.7247728178031,
-8.73055447774162));
#62489=CARTESIAN_POINT('Ctrl Pts',(-16.9473569713774,-20.7854412148401,
-8.73487064048054));
#62490=CARTESIAN_POINT('Ctrl Pts',(-17.0075864459339,-20.8441333452247,
-8.73904620467222));
#62491=CARTESIAN_POINT('Ctrl Pts',(-17.0706676333014,-20.8998122314802,
-8.7432217688639));
#62492=CARTESIAN_POINT('Ctrl Pts',(-17.1362577244092,-20.952204894702,-8.74739733305558));
#62493=CARTESIAN_POINT('Ctrl Pts',(-17.2051606150933,-21.0072437867915,
-8.75178379506812));
#62494=CARTESIAN_POINT('Ctrl Pts',(-17.2768320453054,-21.0586554168247,
-8.75617025708067));
#62495=CARTESIAN_POINT('Ctrl Pts',(-17.3508411420262,-21.1061753813486,
-8.76055671909321));
#62496=CARTESIAN_POINT('Ctrl Pts',(-17.4248502387469,-21.1536953458725,
-8.76494318110575));
#62497=CARTESIAN_POINT('Ctrl Pts',(-17.5011964604718,-21.1973234230529,
-8.76932964311829));
#62498=CARTESIAN_POINT('Ctrl Pts',(-17.5794224113972,-21.2368524223451,
-8.77371610513083));
#62499=CARTESIAN_POINT('Ctrl Pts',(-17.6540490703619,-21.2745626337838,
-8.77790073952388));
#62500=CARTESIAN_POINT('Ctrl Pts',(-17.7306640561251,-21.3086830520783,
-8.78208537391693));
#62501=CARTESIAN_POINT('Ctrl Pts',(-17.8088876493306,-21.3389996101045,
-8.78627000830998));
#62502=CARTESIAN_POINT('Ctrl Pts',(-17.8869999009332,-21.3692730162627,
-8.79044868639392));
#62503=CARTESIAN_POINT('Ctrl Pts',(-17.9667157867298,-21.3957531518832,
-8.79462736447786));
#62504=CARTESIAN_POINT('Ctrl Pts',(-18.047631922491,-21.4182722603509,-8.79880604256181));
#62505=CARTESIAN_POINT('Ctrl Pts',(-18.1299984218322,-21.4411950076538,
-8.80305962044724));
#62506=CARTESIAN_POINT('Ctrl Pts',(-18.2136081930111,-21.4600131107993,
-8.80731319833268));
#62507=CARTESIAN_POINT('Ctrl Pts',(-18.2980154243378,-21.4746013259698,
-8.81156677621812));
#62508=CARTESIAN_POINT('Ctrl Pts',(-18.3807862567781,-21.4889067201227,
-8.81573789019607));
#62509=CARTESIAN_POINT('Ctrl Pts',(-18.4643234304656,-21.4991446900207,
-8.81990900417402));
#62510=CARTESIAN_POINT('Ctrl Pts',(-18.5481939962224,-21.5052481526401,
-8.82408011815197));
#62511=CARTESIAN_POINT('Ctrl Pts',(-18.6320364184009,-21.5113495671838,
-8.82824983247235));
#62512=CARTESIAN_POINT('Ctrl Pts',(-18.7162115520295,-21.5133191964338,
-8.83241954679272));
#62513=CARTESIAN_POINT('Ctrl Pts',(-18.8002812486105,-21.5111418085137,
-8.83658926111309));
#62514=CARTESIAN_POINT('Ctrl Pts',(-18.884347953631,-21.5089644980744,-8.84075882705713));
#62515=CARTESIAN_POINT('Ctrl Pts',(-18.9683087692068,-21.502640476632,-8.84492839300118));
#62516=CARTESIAN_POINT('Ctrl Pts',(-19.0517268423098,-21.4922066163357,
-8.84909795894522));
#62517=CARTESIAN_POINT('Ctrl Pts',(-19.1380777919557,-21.481405914383,-8.85341412168414));
#62518=CARTESIAN_POINT('Ctrl Pts',(-19.2238466000238,-21.4662010579768,
-8.85773028442306));
#62519=CARTESIAN_POINT('Ctrl Pts',(-19.3085579282896,-21.4466910003124,
-8.86204644716198));
#62520=CARTESIAN_POINT('Ctrl Pts',(-19.3905097939473,-21.4278164807242,
-8.86622201135366));
#62521=CARTESIAN_POINT('Ctrl Pts',(-19.4714715762059,-21.404913110059,-8.87039757554534));
#62522=CARTESIAN_POINT('Ctrl Pts',(-19.551028186959,-21.3781213781908,-8.87457313973702));
#62523=CARTESIAN_POINT('Ctrl Pts',(-19.6346030129934,-21.3499764596372,
-8.87895960174956));
#62524=CARTESIAN_POINT('Ctrl Pts',(-19.716626443602,-21.3175402693169,-8.88334606376211));
#62525=CARTESIAN_POINT('Ctrl Pts',(-19.7966429339306,-21.2810319866776,
-8.88773252577465));
#62526=CARTESIAN_POINT('Ctrl Pts',(-19.8766594242592,-21.2445237040383,
-8.89211898778719));
#62527=CARTESIAN_POINT('Ctrl Pts',(-19.954668494674,-21.203943664325,-8.89650544979973));
#62528=CARTESIAN_POINT('Ctrl Pts',(-20.0302483510423,-21.159564316712,-8.90089191181227));
#62529=CARTESIAN_POINT('Ctrl Pts',(-20.102350666183,-21.1172269286686,-8.90507654620531));
#62530=CARTESIAN_POINT('Ctrl Pts',(-20.1725107769709,-21.071274585504,-8.90926118059836));
#62531=CARTESIAN_POINT('Ctrl Pts',(-20.2403431519459,-21.0219107006307,
-8.91344581499141));
#62532=CARTESIAN_POINT('Ctrl Pts',(-20.308078975931,-20.9726170791377,-8.91762449307535));
#62533=CARTESIAN_POINT('Ctrl Pts',(-20.3734932764658,-20.9199218296712,
-8.92180317115929));
#62534=CARTESIAN_POINT('Ctrl Pts',(-20.4362266525525,-20.8640733310571,
-8.92598184924322));
#62535=CARTESIAN_POINT('Ctrl Pts',(-20.50008447932,-20.807223788243,-8.93023542712866));
#62536=CARTESIAN_POINT('Ctrl Pts',(-20.5611639093904,-20.7471070845338,
-8.9344890050141));
#62537=CARTESIAN_POINT('Ctrl Pts',(-20.6191183231211,-20.6840302849064,
-8.93874258289954));
#62538=CARTESIAN_POINT('Ctrl Pts',(-20.675949177453,-20.6221763521241,-8.94291369687749));
#62539=CARTESIAN_POINT('Ctrl Pts',(-20.7297747776525,-20.5574764280246,
-8.94708481085544));
#62540=CARTESIAN_POINT('Ctrl Pts',(-20.7803043703346,-20.4902582435825,
-8.95125592483339));
#62541=CARTESIAN_POINT('Ctrl Pts',(-20.8308170073239,-20.4230626148514,
-8.95542563915376));
#62542=CARTESIAN_POINT('Ctrl Pts',(-20.8780355571481,-20.3533507714295,
-8.95959535347413));
#62543=CARTESIAN_POINT('Ctrl Pts',(-20.9217100507378,-20.2814828821391,
-8.9637650677945));
#62544=CARTESIAN_POINT('Ctrl Pts',(-20.9653829902015,-20.2096175502167,
-8.96793463373855));
#62545=CARTESIAN_POINT('Ctrl Pts',(-21.005511885995,-20.1355967185424,-8.97210419968259));
#62546=CARTESIAN_POINT('Ctrl Pts',(-21.0418912815017,-20.0598076695746,
-8.97627376562663));
#62547=CARTESIAN_POINT('Ctrl Pts',(-21.0795497316757,-19.9813539711409,
-8.98058992836555));
#62548=CARTESIAN_POINT('Ctrl Pts',(-21.113189882732,-19.901005876374,-8.98490609110447));
#62549=CARTESIAN_POINT('Ctrl Pts',(-21.1426376470827,-19.8192166309844,
-8.9892222538434));
#62550=CARTESIAN_POINT('Ctrl Pts',(-21.171126153607,-19.7400916616608,-8.99339781803508));
#62551=CARTESIAN_POINT('Ctrl Pts',(-21.1956911205895,-19.6596184551168,
-8.99757338222676));
#62552=CARTESIAN_POINT('Ctrl Pts',(-21.216225998462,-19.5782220792652,-9.00174894641843));
#62553=CARTESIAN_POINT('Ctrl Pts',(-21.2377980441989,-19.4927145659707,
-9.00613540843098));
#62554=CARTESIAN_POINT('Ctrl Pts',(-21.254922068569,-19.4061887466987,-9.01052187044353));
#62555=CARTESIAN_POINT('Ctrl Pts',(-21.2675357890124,-19.3191463002581,
-9.01490833245607));
#62556=CARTESIAN_POINT('Ctrl Pts',(-21.2801495094559,-19.2321038538175,
-9.01929479446862));
#62557=CARTESIAN_POINT('Ctrl Pts',(-21.288252948244,-19.1445453649661,-9.02368125648116));
#62558=CARTESIAN_POINT('Ctrl Pts',(-21.2918468828523,-19.0569729673898,
-9.02806771849371));
#62559=CARTESIAN_POINT('Ctrl Pts',(-21.2932731600888,-19.022219269613,-9.02980851558631));
#62560=CARTESIAN_POINT('Ctrl Pts',(-21.2939911726516,-18.9874363059255,
-9.03154931267891));
#62561=CARTESIAN_POINT('Ctrl Pts',(-21.2939999191096,-18.9526435515772,
-9.03329010977151));
#62562=CARTESIAN_POINT('Ctrl Pts',(-21.2980343851841,-18.9526308401995,
-9.03329079542781));
#62563=CARTESIAN_POINT('Ctrl Pts',(-21.295285921847,-18.1388728971705,-9.07394170534359));
#62564=CARTESIAN_POINT('Ctrl Pts',(-20.4360628655086,-16.4715240736058,
-9.15698455081984));
#62565=CARTESIAN_POINT('Ctrl Pts',(-18.2953377683469,-16.227376780493,-9.25149015685125));
#62566=CARTESIAN_POINT('Ctrl Pts',(-17.356575497914,-16.7803425229578,-9.30534485296688));
#62567=CARTESIAN_POINT('Ctrl Pts',(-17.1750494511459,-16.9226083978003,
-9.31680761352203));
#62568=CARTESIAN_POINT('',(-21.293999998394,-18.9519093211995,-8.96670989026365));
#62569=CARTESIAN_POINT('Ctrl Pts',(-21.293999998394,-18.9519093211995,-8.96670989026365));
#62570=CARTESIAN_POINT('Ctrl Pts',(-21.2939968622717,-18.8633718327361,
-8.97108917708312));
#62571=CARTESIAN_POINT('Ctrl Pts',(-21.2893963356695,-18.7749281972304,
-8.97546846390259));
#62572=CARTESIAN_POINT('Ctrl Pts',(-21.2802532223815,-18.6870575014991,
-8.97984775072206));
#62573=CARTESIAN_POINT('Ctrl Pts',(-21.2710840473103,-18.5989363367038,
-8.98423952038192));
#62574=CARTESIAN_POINT('Ctrl Pts',(-21.2573464424812,-18.5113917635122,
-8.98863129004178));
#62575=CARTESIAN_POINT('Ctrl Pts',(-21.2391468026208,-18.4248951742595,
-8.99302305970165));
#62576=CARTESIAN_POINT('Ctrl Pts',(-21.2209205771356,-18.3382722327336,
-8.99742124475991));
#62577=CARTESIAN_POINT('Ctrl Pts',(-21.1982194166656,-18.2527007028949,
-9.00181942981817));
#62578=CARTESIAN_POINT('Ctrl Pts',(-21.1711995861976,-18.1686366251616,
-9.00621761487642));
#62579=CARTESIAN_POINT('Ctrl Pts',(-21.1441046030878,-18.0843387325816,
-9.01062803299538));
#62580=CARTESIAN_POINT('Ctrl Pts',(-21.1126670698913,-18.0015570394273,
-9.01503845111433));
#62581=CARTESIAN_POINT('Ctrl Pts',(-21.0770917883152,-17.9207285170577,
-9.01944886923329));
#62582=CARTESIAN_POINT('Ctrl Pts',(-21.0501146625114,-17.859435362938,-9.02279333761614));
#62583=CARTESIAN_POINT('Ctrl Pts',(-21.0207591774504,-17.7992649146786,
-9.02613780599899));
#62584=CARTESIAN_POINT('Ctrl Pts',(-20.9891316170539,-17.7403971815138,
-9.02948227438184));
#62585=CARTESIAN_POINT('Ctrl Pts',(-20.949558877278,-17.6667412480012,-9.03366690877489));
#62586=CARTESIAN_POINT('Ctrl Pts',(-20.9063001320241,-17.5948890389388,
-9.03785154316794));
#62587=CARTESIAN_POINT('Ctrl Pts',(-20.8595440286336,-17.5252335221418,
-9.04203617756098));
#62588=CARTESIAN_POINT('Ctrl Pts',(-20.812854476769,-17.4556771513512,-9.04621485564493));
#62589=CARTESIAN_POINT('Ctrl Pts',(-20.7626777089518,-17.3883116408712,
-9.05039353372888));
#62590=CARTESIAN_POINT('Ctrl Pts',(-20.7092482964897,-17.3235055519854,
-9.05457221181283));
#62591=CARTESIAN_POINT('Ctrl Pts',(-20.6548612002084,-17.2575378605317,
-9.05882578969826));
#62592=CARTESIAN_POINT('Ctrl Pts',(-20.5971039332157,-17.1942226731584,
-9.06307936758369));
#62593=CARTESIAN_POINT('Ctrl Pts',(-20.5362701954422,-17.1339180044286,
-9.06733294546913));
#62594=CARTESIAN_POINT('Ctrl Pts',(-20.4766158383827,-17.0747824593771,
-9.07150405944708));
#62595=CARTESIAN_POINT('Ctrl Pts',(-20.4140035745828,-17.0185420838701,
-9.07567517342503));
#62596=CARTESIAN_POINT('Ctrl Pts',(-20.3487498736144,-16.9654998500724,
-9.07984628740299));
#62597=CARTESIAN_POINT('Ctrl Pts',(-20.2835180691556,-16.9124754151086,
-9.08401600172336));
#62598=CARTESIAN_POINT('Ctrl Pts',(-20.2156469445306,-16.8626472804563,
-9.08818571604373));
#62599=CARTESIAN_POINT('Ctrl Pts',(-20.1454869304126,-16.8162788933771,
-9.0923554303641));
#62600=CARTESIAN_POINT('Ctrl Pts',(-20.0753294128889,-16.7699121562841,
-9.09652499630815));
#62601=CARTESIAN_POINT('Ctrl Pts',(-20.0028835520724,-16.7270051749182,
-9.10069456225219));
#62602=CARTESIAN_POINT('Ctrl Pts',(-19.9285285607302,-16.687777944282,-9.10486412819624));
#62603=CARTESIAN_POINT('Ctrl Pts',(-19.8515593396191,-16.6471715326087,
-9.10918029093515));
#62604=CARTESIAN_POINT('Ctrl Pts',(-19.7725447065605,-16.6105086923156,
-9.11349645367407));
#62605=CARTESIAN_POINT('Ctrl Pts',(-19.6919309796755,-16.577980573336,-9.11781261641299));
#62606=CARTESIAN_POINT('Ctrl Pts',(-19.6139432364648,-16.5465120544109,
-9.12198818060467));
#62607=CARTESIAN_POINT('Ctrl Pts',(-19.5344594409715,-16.5189131263823,
-9.12616374479635));
#62608=CARTESIAN_POINT('Ctrl Pts',(-19.4539003149003,-16.4953063812094,
-9.13033930898803));
#62609=CARTESIAN_POINT('Ctrl Pts',(-19.3692723388824,-16.4705073154575,
-9.13472577100057));
#62610=CARTESIAN_POINT('Ctrl Pts',(-19.2834581156084,-16.4501144565313,
-9.13911223301311));
#62611=CARTESIAN_POINT('Ctrl Pts',(-19.1969566012277,-16.4342090663878,
-9.14349869502565));
#62612=CARTESIAN_POINT('Ctrl Pts',(-19.1104550868471,-16.4183036762444,
-9.14788515703819));
#62613=CARTESIAN_POINT('Ctrl Pts',(-19.0232668665414,-16.406885754803,-9.15227161905072));
#62614=CARTESIAN_POINT('Ctrl Pts',(-18.9358937423135,-16.3999735665917,
-9.15665808106326));
#62615=CARTESIAN_POINT('Ctrl Pts',(-18.8525619577046,-16.3933810933994,
-9.16084165250876));
#62616=CARTESIAN_POINT('Ctrl Pts',(-18.768751898504,-16.3908622168773,-9.16502522395427));
#62617=CARTESIAN_POINT('Ctrl Pts',(-18.6848957690259,-16.3924709858061,
-9.16920879539977));
#62618=CARTESIAN_POINT('Ctrl Pts',(-18.6011496144028,-16.3940776448816,
-9.17338688021399));
#62619=CARTESIAN_POINT('Ctrl Pts',(-18.517357964957,-16.3998011941734,-9.17756496502821));
#62620=CARTESIAN_POINT('Ctrl Pts',(-18.4339575045038,-16.4096439075345,
-9.18174304984243));
#62621=CARTESIAN_POINT('Ctrl Pts',(-18.3506413936532,-16.4194766661668,
-9.18591690902299));
#62622=CARTESIAN_POINT('Ctrl Pts',(-18.2677161403437,-16.4334202620682,
-9.19009076820354));
#62623=CARTESIAN_POINT('Ctrl Pts',(-18.185616418364,-16.4514249766519,-9.1942646273841));
#62624=CARTESIAN_POINT('Ctrl Pts',(-18.1035750976745,-16.4694168836581,
-9.19843551750757));
#62625=CARTESIAN_POINT('Ctrl Pts',(-18.0223585896044,-16.4914640715327,
-9.20260640763105));
#62626=CARTESIAN_POINT('Ctrl Pts',(-17.9423930915556,-16.517465444381,-9.20677729775453));
#62627=CARTESIAN_POINT('Ctrl Pts',(-17.8624446940949,-16.5434612568466,
-9.21094729593491));
#62628=CARTESIAN_POINT('Ctrl Pts',(-17.7837472149657,-16.5734094406324,
-9.21511729411528));
#62629=CARTESIAN_POINT('Ctrl Pts',(-17.7067122821122,-16.6071588657914,
-9.21928729229566));
#62630=CARTESIAN_POINT('Ctrl Pts',(-17.6296873849781,-16.6409038942468,
-9.22345674722987));
#62631=CARTESIAN_POINT('Ctrl Pts',(-17.5543250225282,-16.678448989543,-9.22762620216409));
#62632=CARTESIAN_POINT('Ctrl Pts',(-17.481015873204,-16.7195952925159,-9.2317956570983));
#62633=CARTESIAN_POINT('Ctrl Pts',(-17.4076680317964,-16.7607633122349,
-9.23596731264321));
#62634=CARTESIAN_POINT('Ctrl Pts',(-17.3363759656345,-16.805536104046,-9.24013896818811));
#62635=CARTESIAN_POINT('Ctrl Pts',(-17.267504027417,-16.8536698156873,-9.24431062373302));
#62636=CARTESIAN_POINT('Ctrl Pts',(-17.2359729692538,-16.8757064666173,
-9.24622049758045));
#62637=CARTESIAN_POINT('Ctrl Pts',(-17.2049487630074,-16.8984469736806,
-9.24813037142788));
#62638=CARTESIAN_POINT('Ctrl Pts',(-17.1744641548915,-16.9218650419685,
-9.25004024527531));
#62639=CARTESIAN_POINT('Ctrl Pts',(-17.1744641548914,-16.9218650419685,
-8.45013430174985));
#62640=CARTESIAN_POINT('Ctrl Pts',(-17.1077839597158,-16.9730883136647,
-8.45430378660374));
#62641=CARTESIAN_POINT('Ctrl Pts',(-17.0436166359205,-17.0276105362849,
-8.45847327145763));
#62642=CARTESIAN_POINT('Ctrl Pts',(-16.9822966765068,-17.0851482473258,
-8.46264275631152));
#62643=CARTESIAN_POINT('Ctrl Pts',(-16.9209698311314,-17.1426924195984,
-8.46681270938022));
#62644=CARTESIAN_POINT('Ctrl Pts',(-16.8624913196026,-17.2032524369424,
-8.47098266244893));
#62645=CARTESIAN_POINT('Ctrl Pts',(-16.8071595240486,-17.2665072589194,
-8.47515261551763));
#62646=CARTESIAN_POINT('Ctrl Pts',(-16.7517686221848,-17.3298296507098,
-8.47932702299695));
#62647=CARTESIAN_POINT('Ctrl Pts',(-16.6995314504634,-17.3958522471909,
-8.48350143047628));
#62648=CARTESIAN_POINT('Ctrl Pts',(-16.650706396123,-17.464220527079,-8.4876758379556));
#62649=CARTESIAN_POINT('Ctrl Pts',(-16.6018533425747,-17.5326280134299,
-8.49185263928996));
#62650=CARTESIAN_POINT('Ctrl Pts',(-16.5564165506132,-17.6033834741459,
-8.49602944062433));
#62651=CARTESIAN_POINT('Ctrl Pts',(-16.5146099894966,-17.6761050273326,
-8.50020624195869));
#62652=CARTESIAN_POINT('Ctrl Pts',(-16.4727322757655,-17.7489503488588,
-8.50439015199387));
#62653=CARTESIAN_POINT('Ctrl Pts',(-16.4344973396758,-17.8237680350171,
-8.50857406202906));
#62654=CARTESIAN_POINT('Ctrl Pts',(-16.4000721519639,-17.9001536233072,
-8.51275797206425));
#62655=CARTESIAN_POINT('Ctrl Pts',(-16.3780730306812,-17.9489671791,-8.5154316639282));
#62656=CARTESIAN_POINT('Ctrl Pts',(-16.3576287294878,-17.9984206275095,
-8.51810535579216));
#62657=CARTESIAN_POINT('Ctrl Pts',(-16.3387721302027,-18.0484052613331,
-8.52077904765611));
#62658=CARTESIAN_POINT('Ctrl Pts',(-16.3092593897976,-18.1266369456353,
-8.52496368204916));
#62659=CARTESIAN_POINT('Ctrl Pts',(-16.2835285016033,-18.2064616309202,
-8.5291483164422));
#62660=CARTESIAN_POINT('Ctrl Pts',(-16.2617516946765,-18.2874788815808,
-8.53333295083525));
#62661=CARTESIAN_POINT('Ctrl Pts',(-16.2400058843389,-18.3683808142131,
-8.5375116289192));
#62662=CARTESIAN_POINT('Ctrl Pts',(-16.2222030943944,-18.450471500049,-8.54169030700315));
#62663=CARTESIAN_POINT('Ctrl Pts',(-16.2084669780843,-18.5333319271626,
-8.5458689850871));
#62664=CARTESIAN_POINT('Ctrl Pts',(-16.1944846517613,-18.6176775678812,
-8.55012256297253));
#62665=CARTESIAN_POINT('Ctrl Pts',(-16.1847163934876,-18.7028203654208,
-8.55437614085797));
#62666=CARTESIAN_POINT('Ctrl Pts',(-16.1792390499939,-18.7883036704011,
-8.5586297187434));
#62667=CARTESIAN_POINT('Ctrl Pts',(-16.1738678954921,-18.8721297147074,
-8.56280083272135));
#62668=CARTESIAN_POINT('Ctrl Pts',(-16.1726227957354,-18.9562827012374,
-8.56697194669931));
#62669=CARTESIAN_POINT('Ctrl Pts',(-16.1755241458591,-19.0403249895438,
-8.57114306067726));
#62670=CARTESIAN_POINT('Ctrl Pts',(-16.1784245224067,-19.1243390766486,
-8.57531277499763));
#62671=CARTESIAN_POINT('Ctrl Pts',(-16.1854685696706,-19.2082420799258,
-8.579482489318));
#62672=CARTESIAN_POINT('Ctrl Pts',(-16.1966245729686,-19.2915967348155,
-8.58365220363837));
#62673=CARTESIAN_POINT('Ctrl Pts',(-16.2077801792882,-19.374948423589,-8.58782176958242));
#62674=CARTESIAN_POINT('Ctrl Pts',(-16.2230473888477,-19.4577513469169,
-8.59199133552647));
#62675=CARTESIAN_POINT('Ctrl Pts',(-16.2423428203254,-19.5395751007113,
-8.59616090147052));
#62676=CARTESIAN_POINT('Ctrl Pts',(-16.2623166553703,-19.6242756767484,
-8.60047706420944));
#62677=CARTESIAN_POINT('Ctrl Pts',(-16.2866071262492,-19.7079264335903,
-8.60479322694835));
#62678=CARTESIAN_POINT('Ctrl Pts',(-16.3150650107316,-19.790065342138,-8.60910938968727));
#62679=CARTESIAN_POINT('Ctrl Pts',(-16.3425958826201,-19.8695285843793,
-8.61328495387895));
#62680=CARTESIAN_POINT('Ctrl Pts',(-16.3740266108365,-19.9475765433412,
-8.61746051807063));
#62681=CARTESIAN_POINT('Ctrl Pts',(-16.409173118343,-20.0238115367569,-8.6216360822623));
#62682=CARTESIAN_POINT('Ctrl Pts',(-16.4460947923909,-20.1038969784586,
-8.62602254427484));
#62683=CARTESIAN_POINT('Ctrl Pts',(-16.48711720705,-20.1819809787842,-8.63040900628738));
#62684=CARTESIAN_POINT('Ctrl Pts',(-16.531973720249,-20.2576340464641,-8.63479546829992));
#62685=CARTESIAN_POINT('Ctrl Pts',(-16.5768302334481,-20.333287114144,-8.63918193031246));
#62686=CARTESIAN_POINT('Ctrl Pts',(-16.625520460569,-20.4065088081494,-8.643568392325));
#62687=CARTESIAN_POINT('Ctrl Pts',(-16.677728404917,-20.4769088914603,-8.64795485433753));
#62688=CARTESIAN_POINT('Ctrl Pts',(-16.7275341843547,-20.5440697625801,
-8.65213948873058));
#62689=CARTESIAN_POINT('Ctrl Pts',(-16.7807264703943,-20.6089129556999,
-8.65632412312363));
#62690=CARTESIAN_POINT('Ctrl Pts',(-16.8370617843823,-20.6710769052399,
-8.66050875751667));
#62691=CARTESIAN_POINT('Ctrl Pts',(-16.8933169120236,-20.7331523720919,
-8.66468743560061));
#62692=CARTESIAN_POINT('Ctrl Pts',(-16.9527058751385,-20.7925558323524,
-8.66886611368455));
#62693=CARTESIAN_POINT('Ctrl Pts',(-17.0149432821612,-20.8489565100058,
-8.67304479176848));
#62694=CARTESIAN_POINT('Ctrl Pts',(-17.0782962499757,-20.9063681292718,
-8.67729836965392));
#62695=CARTESIAN_POINT('Ctrl Pts',(-17.1446004956328,-20.960667870067,-8.68155194753935));
#62696=CARTESIAN_POINT('Ctrl Pts',(-17.2135136449479,-21.0115439408035,
-8.68580552542479));
#62697=CARTESIAN_POINT('Ctrl Pts',(-17.2810907783904,-21.0614336796322,
-8.68997663940274));
#62698=CARTESIAN_POINT('Ctrl Pts',(-17.3511761736801,-21.1080310270073,
-8.69414775338069));
#62699=CARTESIAN_POINT('Ctrl Pts',(-17.4234128839587,-21.1510819473741,
-8.69831886735864));
#62700=CARTESIAN_POINT('Ctrl Pts',(-17.4956253545116,-21.1941184215888,
-8.70248858167901));
#62701=CARTESIAN_POINT('Ctrl Pts',(-17.5699873115125,-21.2336105969121,
-8.70665829599938));
#62702=CARTESIAN_POINT('Ctrl Pts',(-17.6461139181095,-21.26934845736,-8.71082801031975));
#62703=CARTESIAN_POINT('Ctrl Pts',(-17.7222378157951,-21.3050850461015,
-8.71499757626379));
#62704=CARTESIAN_POINT('Ctrl Pts',(-17.8001258214361,-21.337067390866,-8.71916714220783));
#62705=CARTESIAN_POINT('Ctrl Pts',(-17.8793709005793,-21.3651326325802,
-8.72333670815187));
#62706=CARTESIAN_POINT('Ctrl Pts',(-17.9614021389459,-21.3941846135708,
-8.7276528708908));
#62707=CARTESIAN_POINT('Ctrl Pts',(-18.0448871586123,-21.4190387397285,
-8.73196903362972));
#62708=CARTESIAN_POINT('Ctrl Pts',(-18.1293566950608,-21.4395703957461,
-8.73628519636865));
#62709=CARTESIAN_POINT('Ctrl Pts',(-18.2110746452441,-21.4594332352284,
-8.74046076056033));
#62710=CARTESIAN_POINT('Ctrl Pts',(-18.2937134844264,-21.4752508467085,
-8.74463632475201));
#62711=CARTESIAN_POINT('Ctrl Pts',(-18.3768391873469,-21.4869627519759,
-8.74881188894369));
#62712=CARTESIAN_POINT('Ctrl Pts',(-18.4641633719094,-21.4992661977359,
-8.75319835095624));
#62713=CARTESIAN_POINT('Ctrl Pts',(-18.5520243141257,-21.5070382273415,
-8.75758481296878));
#62714=CARTESIAN_POINT('Ctrl Pts',(-18.6399165515108,-21.5102705690994,
-8.76197127498133));
#62715=CARTESIAN_POINT('Ctrl Pts',(-18.7278087888959,-21.5135029108574,
-8.76635773699387));
#62716=CARTESIAN_POINT('Ctrl Pts',(-18.8157317424276,-21.5121956494501,
-8.77074419900642));
#62717=CARTESIAN_POINT('Ctrl Pts',(-18.9031862415111,-21.5064032601928,
-8.77513066101897));
#62718=CARTESIAN_POINT('Ctrl Pts',(-18.9866168294529,-21.5008773873516,
-8.77931529541201));
#62719=CARTESIAN_POINT('Ctrl Pts',(-19.0699316687706,-21.4912494832414,
-8.78349992980506));
#62720=CARTESIAN_POINT('Ctrl Pts',(-19.1526949496532,-21.4775285662876,
-8.78768456419811));
#62721=CARTESIAN_POINT('Ctrl Pts',(-19.2353404272498,-21.4638271793609,
-8.79186324228205));
#62722=CARTESIAN_POINT('Ctrl Pts',(-19.317435455861,-21.4460444262517,-8.79604192036601));
#62723=CARTESIAN_POINT('Ctrl Pts',(-19.3985474281626,-21.424241233319,-8.80022059844995));
#62724=CARTESIAN_POINT('Ctrl Pts',(-19.4811132742735,-21.4020472338226,
-8.80447417633539));
#62725=CARTESIAN_POINT('Ctrl Pts',(-19.5626599937767,-21.3756872759158,
-8.80872775422082));
#62726=CARTESIAN_POINT('Ctrl Pts',(-19.6427400986363,-21.3452804752328,
-8.81298133210625));
#62727=CARTESIAN_POINT('Ctrl Pts',(-19.7212676943997,-21.315463169715,-8.8171524460842));
#62728=CARTESIAN_POINT('Ctrl Pts',(-19.7983845845478,-21.2817547038762,
-8.82132356006215));
#62729=CARTESIAN_POINT('Ctrl Pts',(-19.8736839568166,-21.2443177089083,
-8.8254946740401));
#62730=CARTESIAN_POINT('Ctrl Pts',(-19.9489580616539,-21.2068932762857,
-8.82966438836047));
#62731=CARTESIAN_POINT('Ctrl Pts',(-20.0224154482671,-21.1657430039569,
-8.83383410268084));
#62732=CARTESIAN_POINT('Ctrl Pts',(-20.0936712215604,-21.1210768011439,
-8.83800381700122));
#62733=CARTESIAN_POINT('Ctrl Pts',(-20.1649244592675,-21.076412187746,-8.84217338294525));
#62734=CARTESIAN_POINT('Ctrl Pts',(-20.2339758500892,-21.0282321376739,
-8.8463429488893));
#62735=CARTESIAN_POINT('Ctrl Pts',(-20.3004681352884,-20.9767907499606,
-8.85051251483334));
#62736=CARTESIAN_POINT('Ctrl Pts',(-20.3692982072082,-20.9235407465151,
-8.85482867757226));
#62737=CARTESIAN_POINT('Ctrl Pts',(-20.4353854517828,-20.8667961238598,
-8.85914484031118));
#62738=CARTESIAN_POINT('Ctrl Pts',(-20.4983710832766,-20.8068840072892,
-8.86346100305011));
#62739=CARTESIAN_POINT('Ctrl Pts',(-20.5593049644494,-20.7489235216143,
-8.86763656724179));
#62740=CARTESIAN_POINT('Ctrl Pts',(-20.6173359087927,-20.6879991088313,
-8.87181213143346));
#62741=CARTESIAN_POINT('Ctrl Pts',(-20.6721781340605,-20.6244429797902,
-8.87598769562514));
#62742=CARTESIAN_POINT('Ctrl Pts',(-20.7297903097517,-20.5576767817616,
-8.88037415763769));
#62743=CARTESIAN_POINT('Ctrl Pts',(-20.7838828183068,-20.4880064858706,
-8.88476061965023));
#62744=CARTESIAN_POINT('Ctrl Pts',(-20.8341751072844,-20.4158526287653,
-8.88914708166277));
#62745=CARTESIAN_POINT('Ctrl Pts',(-20.884467396262,-20.34369877166,-8.89353354367531));
#62746=CARTESIAN_POINT('Ctrl Pts',(-20.930959223453,-20.2690618860433,-8.89792000568786));
#62747=CARTESIAN_POINT('Ctrl Pts',(-20.9734262024012,-20.1923911818451,
-8.9023064677004));
#62748=CARTESIAN_POINT('Ctrl Pts',(-21.0159038253685,-20.1157012607291,
-8.90669402914565));
#62749=CARTESIAN_POINT('Ctrl Pts',(-21.0545007977188,-20.0367143701651,
-8.9110815905909));
#62750=CARTESIAN_POINT('Ctrl Pts',(-21.0889748257324,-19.9558394145314,
-8.91546915203614));
#62751=CARTESIAN_POINT('Ctrl Pts',(-21.1233545067051,-19.8751857940067,
-8.91984470579146));
#62752=CARTESIAN_POINT('Ctrl Pts',(-21.1536335666925,-19.7926547636184,
-8.92422025954678));
#62753=CARTESIAN_POINT('Ctrl Pts',(-21.1796158858339,-19.7086788876113,
-8.92859581330209));
#62754=CARTESIAN_POINT('Ctrl Pts',(-21.2055560013419,-19.6248394154053,
-8.9329642597524));
#62755=CARTESIAN_POINT('Ctrl Pts',(-21.227213143681,-19.5395601416149,-8.9373327062027));
#62756=CARTESIAN_POINT('Ctrl Pts',(-21.2444392039472,-19.4532933305808,
-8.94170115265301));
#62757=CARTESIAN_POINT('Ctrl Pts',(-21.2616295048391,-19.3672055997974,
-8.94606053069709));
#62758=CARTESIAN_POINT('Ctrl Pts',(-21.2744069696189,-19.2801348014838,
-8.95041990874118));
#62759=CARTESIAN_POINT('Ctrl Pts',(-21.2826736357251,-19.1925466660746,
-8.95477928678526));
#62760=CARTESIAN_POINT('Ctrl Pts',(-21.2902149496553,-19.1126438833585,
-8.95875615459968));
#62761=CARTESIAN_POINT('Ctrl Pts',(-21.2940028463113,-19.0323109723971,
-8.9627330224141));
#62762=CARTESIAN_POINT('Ctrl Pts',(-21.293999998394,-18.95190932191,-8.96670989022851));
#62763=CARTESIAN_POINT('Origin',(-18.734,-18.952,1.76670989022851));
#62764=CARTESIAN_POINT('',(-17.1732300669911,-16.9202871232308,-7.65021348292981));
#62765=CARTESIAN_POINT('',(-17.1756294774617,-16.9234129801347,-7.71658757349708));
#62766=CARTESIAN_POINT('',(-17.1744641548914,-16.9218650419685,1.76670989022851));
#62767=CARTESIAN_POINT('',(-21.2939989173812,-18.9496456407966,-8.23329012251171));
#62768=CARTESIAN_POINT('Ctrl Pts',(-17.175629477462,-16.9234129801345,-7.71658757349706));
#62769=CARTESIAN_POINT('Ctrl Pts',(-16.9627571704335,-17.084021412314,-7.72982826622449));
#62770=CARTESIAN_POINT('Ctrl Pts',(-16.1737486124771,-17.8922292135007,
-7.7854608945124));
#62771=CARTESIAN_POINT('Ctrl Pts',(-15.939111508382,-20.1147077358832,-7.88348545836079));
#62772=CARTESIAN_POINT('Ctrl Pts',(-18.1988330721293,-21.9314105656949,
-8.01066126504222));
#62773=CARTESIAN_POINT('Ctrl Pts',(-20.7208249517526,-21.0909115417432,
-8.12726281551247));
#62774=CARTESIAN_POINT('Ctrl Pts',(-21.2877697529773,-19.5894613481947,
-8.20147243042223));
#62775=CARTESIAN_POINT('Ctrl Pts',(-21.2935816048406,-18.9496462807751,
-8.23329010977151));
#62776=CARTESIAN_POINT('Ctrl Pts',(-21.2939989173812,-18.9496456407966,
-8.23329012251171));
#62777=CARTESIAN_POINT('Ctrl Pts',(-21.2938985191548,-18.8404782076697,
-8.23871812867059));
#62778=CARTESIAN_POINT('Ctrl Pts',(-21.2868114602984,-18.7316228556169,
-8.24414613482947));
#62779=CARTESIAN_POINT('Ctrl Pts',(-21.272879163598,-18.6238345041783,-8.24957414098835));
#62780=CARTESIAN_POINT('Ctrl Pts',(-21.2596700733063,-18.5216412981934,
-8.25472038679393));
#62781=CARTESIAN_POINT('Ctrl Pts',(-21.2403084403045,-18.4204066645113,
-8.25986663259951));
#62782=CARTESIAN_POINT('Ctrl Pts',(-21.2149532278239,-18.3207543415199,
-8.26501287840509));
#62783=CARTESIAN_POINT('Ctrl Pts',(-21.1943358111288,-18.2397227402535,
-8.26919751279814));
#62784=CARTESIAN_POINT('Ctrl Pts',(-21.1697059337058,-18.1595514977396,
-8.27338214719119));
#62785=CARTESIAN_POINT('Ctrl Pts',(-21.1411517779373,-18.0806675043515,
-8.27756678158423));
#62786=CARTESIAN_POINT('Ctrl Pts',(-21.1126382654753,-18.001895792564,-8.28174545966817));
#62787=CARTESIAN_POINT('Ctrl Pts',(-21.0802117249138,-17.9244081193636,
-8.28592413775212));
#62788=CARTESIAN_POINT('Ctrl Pts',(-21.0440107968602,-17.8486187792111,
-8.29010281583606));
#62789=CARTESIAN_POINT('Ctrl Pts',(-21.0071609931883,-17.7714709696052,
-8.29435639372149));
#62790=CARTESIAN_POINT('Ctrl Pts',(-20.9664002781983,-17.6960834444032,
-8.29860997160693));
#62791=CARTESIAN_POINT('Ctrl Pts',(-20.9219272181895,-17.6228745401936,
-8.30286354949236));
#62792=CARTESIAN_POINT('Ctrl Pts',(-20.8783163552311,-17.5510849334477,
-8.30703466347032));
#62793=CARTESIAN_POINT('Ctrl Pts',(-20.8311360546879,-17.481390639162,-8.31120577744827));
#62794=CARTESIAN_POINT('Ctrl Pts',(-20.7806202689679,-17.4141620778997,
-8.31537689142622));
#62795=CARTESIAN_POINT('Ctrl Pts',(-20.7301214343076,-17.3469560758303,
-8.31954660574659));
#62796=CARTESIAN_POINT('Ctrl Pts',(-20.6762896134472,-17.282214531026,-8.32371632006697));
#62797=CARTESIAN_POINT('Ctrl Pts',(-20.6194012584856,-17.2202777086088,
-8.32788603438734));
#62798=CARTESIAN_POINT('Ctrl Pts',(-20.5625149278558,-17.1583430901696,
-8.33205560033139));
#62799=CARTESIAN_POINT('Ctrl Pts',(-20.5025725911955,-17.0992133339121,
-8.33622516627543));
#62800=CARTESIAN_POINT('Ctrl Pts',(-20.4398891227942,-17.0431934878746,
-8.34039473221947));
#62801=CARTESIAN_POINT('Ctrl Pts',(-20.3750017809723,-16.9852040531583,
-8.34471089495839));
#62802=CARTESIAN_POINT('Ctrl Pts',(-20.307177357872,-16.9305476379184,-8.34902705769732));
#62803=CARTESIAN_POINT('Ctrl Pts',(-20.2368028123898,-16.8795175013831,
-8.35334322043624));
#62804=CARTESIAN_POINT('Ctrl Pts',(-20.1687207103246,-16.8301496661781,
-8.35751878462792));
#62805=CARTESIAN_POINT('Ctrl Pts',(-20.0982524952705,-16.7841757035315,
-8.3616943488196));
#62806=CARTESIAN_POINT('Ctrl Pts',(-20.0257768405865,-16.7418161628217,
-8.36586991301128));
#62807=CARTESIAN_POINT('Ctrl Pts',(-19.949640612879,-16.6973171424109,-8.37025637502382));
#62808=CARTESIAN_POINT('Ctrl Pts',(-19.8712893431908,-16.6568075367651,
-8.37464283703636));
#62809=CARTESIAN_POINT('Ctrl Pts',(-19.7911876038235,-16.6204866780733,
-8.3790292990489));
#62810=CARTESIAN_POINT('Ctrl Pts',(-19.7110858644562,-16.5841658193814,
-8.38341576106144));
#62811=CARTESIAN_POINT('Ctrl Pts',(-19.6292342232969,-16.5520338488593,
-8.38780222307399));
#62812=CARTESIAN_POINT('Ctrl Pts',(-19.5461152252309,-16.524229652346,-8.39218868508653));
#62813=CARTESIAN_POINT('Ctrl Pts',(-19.4668195289802,-16.4977043913044,
-8.39637337892856));
#62814=CARTESIAN_POINT('Ctrl Pts',(-19.3860753481911,-16.4750187798306,
-8.40055807277059));
#62815=CARTESIAN_POINT('Ctrl Pts',(-19.304289379044,-16.4563297445076,-8.40474276661262));
#62816=CARTESIAN_POINT('Ctrl Pts',(-19.2226201402028,-16.4376673834031,
-8.40892148778481));
#62817=CARTESIAN_POINT('Ctrl Pts',(-19.1399125111903,-16.4229903695736,
-8.41310020895699));
#62818=CARTESIAN_POINT('Ctrl Pts',(-19.0565899050055,-16.4124063803064,
-8.41727893012918));
#62819=CARTESIAN_POINT('Ctrl Pts',(-18.973365253887,-16.4018348337053,-8.42145273874608));
#62820=CARTESIAN_POINT('Ctrl Pts',(-18.8895275166888,-16.3953468042853,
-8.42562654736298));
#62821=CARTESIAN_POINT('Ctrl Pts',(-18.8055104987655,-16.392998974489,-8.42980035597989));
#62822=CARTESIAN_POINT('Ctrl Pts',(-18.7215478255247,-16.3906526633382,
-8.43397146485441));
#62823=CARTESIAN_POINT('Ctrl Pts',(-18.6374065603179,-16.3924412477093,
-8.43814257372892));
#62824=CARTESIAN_POINT('Ctrl Pts',(-18.5535247699726,-16.3983695076722,
-8.44231368260344));
#62825=CARTESIAN_POINT('Ctrl Pts',(-18.4696720738781,-16.4042957114285,
-8.44648334473622));
#62826=CARTESIAN_POINT('Ctrl Pts',(-18.3860791323488,-16.4143587064509,
-8.45065300686901));
#62827=CARTESIAN_POINT('Ctrl Pts',(-18.3031817775233,-16.4285112127885,
-8.45482266900179));
#62828=CARTESIAN_POINT('Ctrl Pts',(-18.2202883084439,-16.4426630557389,
-8.45899213568505));
#62829=CARTESIAN_POINT('Ctrl Pts',(-18.1380908144806,-16.4609039503763,
-8.46316160236831));
#62830=CARTESIAN_POINT('Ctrl Pts',(-18.0570164290525,-16.4831352315959,
-8.46733106905157));
#62831=CARTESIAN_POINT('Ctrl Pts',(-17.9758686662696,-16.5053866335059,
-8.47150430936117));
#62832=CARTESIAN_POINT('Ctrl Pts',(-17.8958464874503,-16.5316355155317,
-8.47567754967078));
#62833=CARTESIAN_POINT('Ctrl Pts',(-17.8173628033139,-16.5617330170771,
-8.47985078998038));
#62834=CARTESIAN_POINT('Ctrl Pts',(-17.738845097665,-16.5918435654428,-8.48402583932774));
#62835=CARTESIAN_POINT('Ctrl Pts',(-17.6618676372617,-16.6258058721945,
-8.48820088867509));
#62836=CARTESIAN_POINT('Ctrl Pts',(-17.5868220329166,-16.6634234310737,
-8.49237593802245));
#62837=CARTESIAN_POINT('Ctrl Pts',(-17.5116490487983,-16.7011048406762,
-8.49655807395194));
#62838=CARTESIAN_POINT('Ctrl Pts',(-17.4384148750597,-16.7424536740456,
-8.50074020988144));
#62839=CARTESIAN_POINT('Ctrl Pts',(-17.3674851350989,-16.7872281589035,
-8.50492234581094));
#62840=CARTESIAN_POINT('Ctrl Pts',(-17.3010306427489,-16.829177638249,-8.50884061366708));
#62841=CARTESIAN_POINT('Ctrl Pts',(-17.2365989396928,-16.8741335235576,
-8.51275888152322));
#62842=CARTESIAN_POINT('Ctrl Pts',(-17.1744641548914,-16.9218650419685,
-8.51667714937936));
#62843=CARTESIAN_POINT('',(-21.2939989424941,-18.9543268925436,-8.16670989022853));
#62844=CARTESIAN_POINT('Ctrl Pts',(-21.2939989424941,-18.9543268925437,
-8.16670989022852));
#62845=CARTESIAN_POINT('Ctrl Pts',(-21.2940748047761,-18.8708647825268,
-8.17086478789788));
#62846=CARTESIAN_POINT('Ctrl Pts',(-21.2900646933588,-18.7872780169979,
-8.17501968556725));
#62847=CARTESIAN_POINT('Ctrl Pts',(-21.2819596922617,-18.7040052286649,
-8.17917458323661));
#62848=CARTESIAN_POINT('Ctrl Pts',(-21.2739328413916,-18.621535375116,-8.18328941845664));
#62849=CARTESIAN_POINT('Ctrl Pts',(-21.2618897634889,-18.539373952273,-8.18740425367668));
#62850=CARTESIAN_POINT('Ctrl Pts',(-21.2458740550218,-18.4579466307083,
-8.19151908889671));
#62851=CARTESIAN_POINT('Ctrl Pts',(-21.2298653109089,-18.3765547174254,
-8.19563213480031));
#62852=CARTESIAN_POINT('Ctrl Pts',(-21.2098874553344,-18.2958967363637,
-8.1997451807039));
#62853=CARTESIAN_POINT('Ctrl Pts',(-21.1860355605651,-18.2163903142807,
-8.20385822660749));
#62854=CARTESIAN_POINT('Ctrl Pts',(-21.1621864189584,-18.1368930694186,
-8.20797079775283));
#62855=CARTESIAN_POINT('Ctrl Pts',(-21.1344642632166,-18.0585475732026,
-8.21208336889816));
#62856=CARTESIAN_POINT('Ctrl Pts',(-21.1030141994635,-17.9817568744174,
-8.2161959400435));
#62857=CARTESIAN_POINT('Ctrl Pts',(-21.0710029255601,-17.9035958852586,
-8.22038189789764));
#62858=CARTESIAN_POINT('Ctrl Pts',(-21.035129571801,-17.8270462022335,-8.22456785575179));
#62859=CARTESIAN_POINT('Ctrl Pts',(-20.9955977974881,-17.7525103575283,
-8.22875381360593));
#62860=CARTESIAN_POINT('Ctrl Pts',(-20.9567081892511,-17.6791852955855,
-8.23287177349703));
#62861=CARTESIAN_POINT('Ctrl Pts',(-20.9142784405326,-17.6078095092631,
-8.23698973338812));
#62862=CARTESIAN_POINT('Ctrl Pts',(-20.8685472200434,-17.5387384653204,
-8.24110769327921));
#62863=CARTESIAN_POINT('Ctrl Pts',(-20.8216832918823,-17.4679566141755,
-8.24532765011488));
#62864=CARTESIAN_POINT('Ctrl Pts',(-20.7713524862055,-17.399595623106,-8.24954760695055));
#62865=CARTESIAN_POINT('Ctrl Pts',(-20.7178552814754,-17.3340017854886,
-8.25376756378622));
#62866=CARTESIAN_POINT('Ctrl Pts',(-20.6643580767453,-17.2684079478711,
-8.25798752062189));
#62867=CARTESIAN_POINT('Ctrl Pts',(-20.6076948817587,-17.2055816046285,
-8.26220747745756));
#62868=CARTESIAN_POINT('Ctrl Pts',(-20.5482046419776,-17.1458268308308,
-8.26642743429323));
#62869=CARTESIAN_POINT('Ctrl Pts',(-20.4892123552949,-17.0865722243692,
-8.27061206868627));
#62870=CARTESIAN_POINT('Ctrl Pts',(-20.427204219073,-17.0301005497847,-8.27479670307932));
#62871=CARTESIAN_POINT('Ctrl Pts',(-20.3624734272386,-16.9767343731088,
-8.27898133747237));
#62872=CARTESIAN_POINT('Ctrl Pts',(-20.2978347716741,-16.9234441565799,
-8.28316001555632));
#62873=CARTESIAN_POINT('Ctrl Pts',(-20.230481510108,-16.8732509480032,-8.28733869364026));
#62874=CARTESIAN_POINT('Ctrl Pts',(-20.1607438576395,-16.8264407877718,
-8.29151737172421));
#62875=CARTESIAN_POINT('Ctrl Pts',(-20.08975620787,-16.7787915890602,-8.29577094960965));
#62876=CARTESIAN_POINT('Ctrl Pts',(-20.0162981861697,-16.7346482555833,
-8.30002452749508));
#62877=CARTESIAN_POINT('Ctrl Pts',(-19.9407536469187,-16.6942698045053,
-8.30427810538052));
#62878=CARTESIAN_POINT('Ctrl Pts',(-19.8666736859741,-16.6546741684936,
-8.30844921935847));
#62879=CARTESIAN_POINT('Ctrl Pts',(-19.7905878123475,-16.6186989652308,
-8.31262033333642));
#62880=CARTESIAN_POINT('Ctrl Pts',(-19.7128859499199,-16.5865439557985,
-8.31679144731437));
#62881=CARTESIAN_POINT('Ctrl Pts',(-19.6352101611027,-16.5543997362902,
-8.32096116163474));
#62882=CARTESIAN_POINT('Ctrl Pts',(-19.5559198851422,-16.5260733404925,
-8.32513087595511));
#62883=CARTESIAN_POINT('Ctrl Pts',(-19.4754262787741,-16.5017169401999,
-8.32930059027548));
#62884=CARTESIAN_POINT('Ctrl Pts',(-19.3949355367137,-16.4773614066125,
-8.33347015621953));
#62885=CARTESIAN_POINT('Ctrl Pts',(-19.3132419899457,-16.4569757200691,
-8.33763972216358));
#62886=CARTESIAN_POINT('Ctrl Pts',(-19.230771941892,-16.4406621816751,-8.34180928810762));
#62887=CARTESIAN_POINT('Ctrl Pts',(-19.1454023486867,-16.4237750793961,
-8.34612545084654));
#62888=CARTESIAN_POINT('Ctrl Pts',(-19.0592011520725,-16.4112519089494,
-8.35044161358546));
#62889=CARTESIAN_POINT('Ctrl Pts',(-18.9726507026517,-16.4031481325656,
-8.35475777632438));
#62890=CARTESIAN_POINT('Ctrl Pts',(-18.8889196250172,-16.3953083358451,
-8.35893334051606));
#62891=CARTESIAN_POINT('Ctrl Pts',(-18.8048621716341,-16.3916044048151,
-8.36310890470774));
#62892=CARTESIAN_POINT('Ctrl Pts',(-18.7209165514642,-16.392033433153,-8.36728446889942));
#62893=CARTESIAN_POINT('Ctrl Pts',(-18.6327310375814,-16.3924841306923,
-8.37167093091196));
#62894=CARTESIAN_POINT('Ctrl Pts',(-18.544669534143,-16.3974962383813,-8.3760573929245));
#62895=CARTESIAN_POINT('Ctrl Pts',(-18.4572333890563,-16.4070048638422,
-8.38044385493705));
#62896=CARTESIAN_POINT('Ctrl Pts',(-18.3697972439697,-16.4165134893032,
-8.38483031694959));
#62897=CARTESIAN_POINT('Ctrl Pts',(-18.2829870179305,-16.4305184650313,
-8.38921677896213));
#62898=CARTESIAN_POINT('Ctrl Pts',(-18.1972887614196,-16.4488937205182,
-8.39360324097467));
#62899=CARTESIAN_POINT('Ctrl Pts',(-18.1155272922731,-16.4664248576231,
-8.39778819867512));
#62900=CARTESIAN_POINT('Ctrl Pts',(-18.0344735156912,-16.4879988204612,
-8.40197315637556));
#62901=CARTESIAN_POINT('Ctrl Pts',(-17.9545574583907,-16.51354365954,-8.40615811407601));
#62902=CARTESIAN_POINT('Ctrl Pts',(-17.8747749678687,-16.5390458045473,
-8.41033607729579));
#62903=CARTESIAN_POINT('Ctrl Pts',(-17.7961268504911,-16.5685054918742,
-8.41451404051556));
#62904=CARTESIAN_POINT('Ctrl Pts',(-17.7190321451558,-16.6017999545501,
-8.41869200373534));
#62905=CARTESIAN_POINT('Ctrl Pts',(-17.6420120287581,-16.6350622049153,
-8.42286592478599));
#62906=CARTESIAN_POINT('Ctrl Pts',(-17.5665427606548,-16.6721516838674,
-8.42703984583664));
#62907=CARTESIAN_POINT('Ctrl Pts',(-17.4930266305908,-16.7128963631808,
-8.43121376688728));
#62908=CARTESIAN_POINT('Ctrl Pts',(-17.4195625033497,-16.7536122210866,
-8.43538473544741));
#62909=CARTESIAN_POINT('Ctrl Pts',(-17.348049170532,-16.7979779202157,-8.43955570400754));
#62910=CARTESIAN_POINT('Ctrl Pts',(-17.2788661013312,-16.8457746234211,
-8.44372667256767));
#62911=CARTESIAN_POINT('Ctrl Pts',(-17.2434387222357,-16.8702504372804,
-8.44586254896173));
#62912=CARTESIAN_POINT('Ctrl Pts',(-17.2086220088753,-16.8956252112277,
-8.44799842535579));
#62913=CARTESIAN_POINT('Ctrl Pts',(-17.1744641548914,-16.9218650419685,
-8.45013430174985));
#62914=CARTESIAN_POINT('Ctrl Pts',(-17.173230066991,-16.9202871232309,-7.65021348292981));
#62915=CARTESIAN_POINT('Ctrl Pts',(-16.6072658842675,-17.3635947026003,
-7.68605039114237));
#62916=CARTESIAN_POINT('Ctrl Pts',(-15.7765851280492,-18.874458207751,-7.76427923491542));
#62917=CARTESIAN_POINT('Ctrl Pts',(-16.9200889756585,-21.3754309612901,
-7.88490001424892));
#62918=CARTESIAN_POINT('Ctrl Pts',(-19.7898862882482,-21.7889693291709,
-8.01207582093036));
#62919=CARTESIAN_POINT('Ctrl Pts',(-21.1940976605954,-20.1719438373811,
-8.10601244625689));
#62920=CARTESIAN_POINT('Ctrl Pts',(-21.2961551338926,-19.1382186499617,
-8.15755713602294));
#62921=CARTESIAN_POINT('Ctrl Pts',(-21.2944496155086,-18.9543273021797,
-8.16670989022852));
#62922=CARTESIAN_POINT('Origin',(-18.734,-18.952,1.76670989022851));
#62923=CARTESIAN_POINT('',(-17.1744641548914,-16.9218650419685,-6.85004462002157));
#62924=CARTESIAN_POINT('',(-17.1744641548914,-16.9218650419685,-6.91673142062773));
#62925=CARTESIAN_POINT('',(-17.1744641548914,-16.9218650419685,1.76670989022851));
#62926=CARTESIAN_POINT('',(-21.29363549648,-18.9525601738873,-7.43329008494618));
#62927=CARTESIAN_POINT('Ctrl Pts',(-17.1744641548914,-16.9218650419685,
-6.91673142062773));
#62928=CARTESIAN_POINT('Ctrl Pts',(-17.1077986118319,-16.9730770580089,
-6.92090111744156));
#62929=CARTESIAN_POINT('Ctrl Pts',(-17.0436334872203,-17.0275952975788,
-6.92507081425539));
#62930=CARTESIAN_POINT('Ctrl Pts',(-16.9823059547924,-17.0851395413732,
-6.92924051106922));
#62931=CARTESIAN_POINT('Ctrl Pts',(-16.9209801805697,-17.1426821354258,
-6.93341008834158));
#62932=CARTESIAN_POINT('Ctrl Pts',(-16.862492171621,-17.2032502457524,-6.93757966561394));
#62933=CARTESIAN_POINT('Ctrl Pts',(-16.807143454622,-17.2665256295233,-6.94174924288631));
#62934=CARTESIAN_POINT('Ctrl Pts',(-16.7501679117016,-17.3316608221585,
-6.94604137361168));
#62935=CARTESIAN_POINT('Ctrl Pts',(-16.696519444733,-17.3996645488824,-6.95033350433705));
#62936=CARTESIAN_POINT('Ctrl Pts',(-16.6464823134451,-17.4701532102405,
-6.95462563506242));
#62937=CARTESIAN_POINT('Ctrl Pts',(-16.5978036071207,-17.5387282215798,
-6.9588012415712));
#62938=CARTESIAN_POINT('Ctrl Pts',(-16.5525428475067,-17.6096545305514,
-6.96297684807997));
#62939=CARTESIAN_POINT('Ctrl Pts',(-16.5109166141274,-17.6825511985679,
-6.96715245458875));
#62940=CARTESIAN_POINT('Ctrl Pts',(-16.4675479521126,-17.7584992414381,
-6.97150284742242));
#62941=CARTESIAN_POINT('Ctrl Pts',(-16.4281250253917,-17.836585719324,-6.97585324025609));
#62942=CARTESIAN_POINT('Ctrl Pts',(-16.3928377730059,-17.9163555499612,
-6.98020363308976));
#62943=CARTESIAN_POINT('Ctrl Pts',(-16.3575505206202,-17.9961253805984,
-6.98455402592343));
#62944=CARTESIAN_POINT('Ctrl Pts',(-16.326399072824,-18.0775780178091,-6.98890441875709));
#62945=CARTESIAN_POINT('Ctrl Pts',(-16.2995147249234,-18.1602415485545,
-6.99325481159076));
#62946=CARTESIAN_POINT('Ctrl Pts',(-16.273654723043,-18.2397554377671,-6.99743944598381));
#62947=CARTESIAN_POINT('Ctrl Pts',(-16.251646255088,-18.3206855701428,-7.00162408037685));
#62948=CARTESIAN_POINT('Ctrl Pts',(-16.233642830573,-18.4026239673095,-7.00580871476989));
#62949=CARTESIAN_POINT('Ctrl Pts',(-16.2156650317043,-18.4844457353098,
-7.00998739285384));
#62950=CARTESIAN_POINT('Ctrl Pts',(-16.2016810508028,-18.5672724719892,
-7.01416607093778));
#62951=CARTESIAN_POINT('Ctrl Pts',(-16.1917950137906,-18.6506798909931,
-7.01834474902173));
#62952=CARTESIAN_POINT('Ctrl Pts',(-16.1817317766699,-18.7355823280388,
-7.02259832690716));
#62953=CARTESIAN_POINT('Ctrl Pts',(-16.1759149888559,-18.8210860111297,
-7.0268519047926));
#62954=CARTESIAN_POINT('Ctrl Pts',(-16.1744002778054,-18.9067312233283,
-7.03110548267803));
#62955=CARTESIAN_POINT('Ctrl Pts',(-16.1729149323844,-18.9907160359655,
-7.03527659665599));
#62956=CARTESIAN_POINT('Ctrl Pts',(-16.1755663524988,-19.0748364579016,
-7.03944771063394));
#62957=CARTESIAN_POINT('Ctrl Pts',(-16.1823546543812,-19.1586543737303,
-7.04361882461189));
#62958=CARTESIAN_POINT('Ctrl Pts',(-16.1891406783834,-19.2424441636479,
-7.04778853893226));
#62959=CARTESIAN_POINT('Ctrl Pts',(-16.2000607901197,-19.3259311909063,
-7.05195825325264));
#62960=CARTESIAN_POINT('Ctrl Pts',(-16.2150630692561,-19.4086801275888,
-7.05612796757301));
#62961=CARTESIAN_POINT('Ctrl Pts',(-16.230064814547,-19.4914261197089,-7.06029753351705));
#62962=CARTESIAN_POINT('Ctrl Pts',(-16.2491483555176,-19.5734336209717,
-7.06446709946108));
#62963=CARTESIAN_POINT('Ctrl Pts',(-16.2722104781215,-19.6542765480702,
-7.06863666540512));
#62964=CARTESIAN_POINT('Ctrl Pts',(-16.2960834365061,-19.7379618127552,
-7.07295282814404));
#62965=CARTESIAN_POINT('Ctrl Pts',(-16.3242198111558,-19.8203985795364,
-7.07726899088297));
#62966=CARTESIAN_POINT('Ctrl Pts',(-16.3564491538595,-19.901132221567,-7.08158515362189));
#62967=CARTESIAN_POINT('Ctrl Pts',(-16.3876286291145,-19.9792359737001,
-7.08576071781356));
#62968=CARTESIAN_POINT('Ctrl Pts',(-16.4226382716202,-20.0557454470086,
-7.08993628200524));
#62969=CARTESIAN_POINT('Ctrl Pts',(-16.4612757941351,-20.1302719058331,
-7.09411184619692));
#62970=CARTESIAN_POINT('Ctrl Pts',(-16.5018648060602,-20.2085625189232,
-7.09849830820946));
#62971=CARTESIAN_POINT('Ctrl Pts',(-16.5464575227362,-20.2846640250238,
-7.10288477022201));
#62972=CARTESIAN_POINT('Ctrl Pts',(-16.5947677080406,-20.3581597352499,
-7.10727123223455));
#62973=CARTESIAN_POINT('Ctrl Pts',(-16.6430778933449,-20.4316554454761,
-7.1116576942471));
#62974=CARTESIAN_POINT('Ctrl Pts',(-16.6951051426578,-20.5025449370743,
-7.11604415625964));
#62975=CARTESIAN_POINT('Ctrl Pts',(-16.7505157350918,-20.5704530178111,
-7.12043061827219));
#62976=CARTESIAN_POINT('Ctrl Pts',(-16.8033768040298,-20.6352365470892,
-7.12461525266524));
#62977=CARTESIAN_POINT('Ctrl Pts',(-16.8595134716063,-20.6975481314175,
-7.12879988705829));
#62978=CARTESIAN_POINT('Ctrl Pts',(-16.918665784363,-20.7570378626327,-7.13298452145133));
#62979=CARTESIAN_POINT('Ctrl Pts',(-16.9777339011242,-20.816442917579,-7.13716319953528));
#62980=CARTESIAN_POINT('Ctrl Pts',(-17.0398088154215,-20.8730337741355,
-7.14134187761923));
#62981=CARTESIAN_POINT('Ctrl Pts',(-17.1045901309625,-20.9264932207236,
-7.14552055570318));
#62982=CARTESIAN_POINT('Ctrl Pts',(-17.170532605027,-20.980910889471,-7.14977413358862));
#62983=CARTESIAN_POINT('Ctrl Pts',(-17.2392791543356,-21.0320834094474,
-7.15402771147406));
#62984=CARTESIAN_POINT('Ctrl Pts',(-17.310473339783,-21.0797151707058,-7.15828128935949));
#62985=CARTESIAN_POINT('Ctrl Pts',(-17.3802872870216,-21.1264234973264,
-7.16245240333745));
#62986=CARTESIAN_POINT('Ctrl Pts',(-17.4524544129442,-21.1697268615306,
-7.1666235173154));
#62987=CARTESIAN_POINT('Ctrl Pts',(-17.5266063947421,-21.2093880220251,
-7.17079463129335));
#62988=CARTESIAN_POINT('Ctrl Pts',(-17.6007334941263,-21.2490358738341,
-7.17496434561372));
#62989=CARTESIAN_POINT('Ctrl Pts',(-17.6768437213087,-21.2850437324073,
-7.1791340599341));
#62990=CARTESIAN_POINT('Ctrl Pts',(-17.7545429309113,-21.3172196197842,
-7.18330377425447));
#62991=CARTESIAN_POINT('Ctrl Pts',(-17.8322393756429,-21.3493943622051,
-7.18747334019852));
#62992=CARTESIAN_POINT('Ctrl Pts',(-17.9115242650163,-21.3777372293231,
-7.19164290614258));
#62993=CARTESIAN_POINT('Ctrl Pts',(-17.9919834625938,-21.4021043770043,
-7.19581247208664));
#62994=CARTESIAN_POINT('Ctrl Pts',(-18.0752715063007,-21.4273282435378,
-7.20012863482555));
#62995=CARTESIAN_POINT('Ctrl Pts',(-18.1598174672116,-21.4482914634568,
-7.20444479756447));
#62996=CARTESIAN_POINT('Ctrl Pts',(-18.2451468157111,-21.4648912758435,
-7.20876096030339));
#62997=CARTESIAN_POINT('Ctrl Pts',(-18.3276965696584,-21.4809503510878,
-7.21293652449507));
#62998=CARTESIAN_POINT('Ctrl Pts',(-18.4109789843022,-21.4929259089215,
-7.21711208868675));
#62999=CARTESIAN_POINT('Ctrl Pts',(-18.4945577002246,-21.5007776256626,
-7.22128765287843));
#63000=CARTESIAN_POINT('Ctrl Pts',(-18.5823577783985,-21.5090259139506,
-7.22567411489096));
#63001=CARTESIAN_POINT('Ctrl Pts',(-18.6704842934734,-21.5127227980494,
-7.23006057690349));
#63002=CARTESIAN_POINT('Ctrl Pts',(-18.7584319418552,-21.5118834114501,
-7.23444703891603));
#63003=CARTESIAN_POINT('Ctrl Pts',(-18.8463795902369,-21.5110440248507,
-7.23883350092856));
#63004=CARTESIAN_POINT('Ctrl Pts',(-18.9341477974438,-21.5056684789459,
-7.24321996294109));
#63005=CARTESIAN_POINT('Ctrl Pts',(-19.0212404493959,-21.4958342957494,
-7.24760642495362));
#63006=CARTESIAN_POINT('Ctrl Pts',(-19.1043258393297,-21.4864525978996,
-7.25179105934668));
#63007=CARTESIAN_POINT('Ctrl Pts',(-19.1871057341709,-21.4729786230522,
-7.25597569373973));
#63008=CARTESIAN_POINT('Ctrl Pts',(-19.2691452086518,-21.455441552275,-7.26016032813278));
#63009=CARTESIAN_POINT('Ctrl Pts',(-19.351067910095,-21.4379294433475,-7.26433900621672));
#63010=CARTESIAN_POINT('Ctrl Pts',(-19.4322518385269,-21.4163658213152,
-7.26851768430066));
#63011=CARTESIAN_POINT('Ctrl Pts',(-19.5122676703939,-21.3908315713103,
-7.2726963623846));
#63012=CARTESIAN_POINT('Ctrl Pts',(-19.5937177285409,-21.3648396382251,
-7.27694994027004));
#63013=CARTESIAN_POINT('Ctrl Pts',(-19.6739569228735,-21.3347333841335,
-7.28120351815547));
#63014=CARTESIAN_POINT('Ctrl Pts',(-19.7525437584804,-21.3006525098577,
-7.2854570960409));
#63015=CARTESIAN_POINT('Ctrl Pts',(-19.8296070349294,-21.267232359833,-7.28962821001886));
#63016=CARTESIAN_POINT('Ctrl Pts',(-19.9050810078233,-21.2299905173577,
-7.29379932399682));
#63017=CARTESIAN_POINT('Ctrl Pts',(-19.9785668286282,-21.1891082694135,
-7.29797043797477));
#63018=CARTESIAN_POINT('Ctrl Pts',(-20.052027990556,-21.1482397399025,-7.30214015229515));
#63019=CARTESIAN_POINT('Ctrl Pts',(-20.1235019236781,-21.1037334544493,
-7.30630986661552));
#63020=CARTESIAN_POINT('Ctrl Pts',(-20.1926138614934,-21.0558169129131,
-7.31047958093589));
#63021=CARTESIAN_POINT('Ctrl Pts',(-20.2617233400094,-21.0079020764531,
-7.31464914687994));
#63022=CARTESIAN_POINT('Ctrl Pts',(-20.3284706127605,-20.9565774880019,
-7.31881871282399));
#63023=CARTESIAN_POINT('Ctrl Pts',(-20.3925105653949,-20.9021135106638,
-7.32298827876803));
#63024=CARTESIAN_POINT('Ctrl Pts',(-20.458802083762,-20.8457346470711,-7.32730444150695));
#63025=CARTESIAN_POINT('Ctrl Pts',(-20.5221919593126,-20.7859918669766,
-7.33162060424587));
#63026=CARTESIAN_POINT('Ctrl Pts',(-20.5823369324963,-20.7232285521553,
-7.33593676698479));
#63027=CARTESIAN_POINT('Ctrl Pts',(-20.6405226895047,-20.6625097457128,
-7.34011233117647));
#63028=CARTESIAN_POINT('Ctrl Pts',(-20.6956714299404,-20.5989645570462,
-7.34428789536814));
#63029=CARTESIAN_POINT('Ctrl Pts',(-20.7475130548916,-20.5329380689265,
-7.34846345955982));
#63030=CARTESIAN_POINT('Ctrl Pts',(-20.8019730770774,-20.4635767398549,
-7.35284992157236));
#63031=CARTESIAN_POINT('Ctrl Pts',(-20.8527827827185,-20.3914773402459,
-7.3572363835849));
#63032=CARTESIAN_POINT('Ctrl Pts',(-20.8996813854343,-20.3170729419278,
-7.36162284559744));
#63033=CARTESIAN_POINT('Ctrl Pts',(-20.94657998815,-20.2426685436098,-7.36600930760998));
#63034=CARTESIAN_POINT('Ctrl Pts',(-20.9895672706481,-20.1659596899256,
-7.37039576962251));
#63035=CARTESIAN_POINT('Ctrl Pts',(-21.0284398795321,-20.0874054955005,
-7.37478223163505));
#63036=CARTESIAN_POINT('Ctrl Pts',(-21.0682036058612,-20.0070505211677,
-7.37926924910127));
#63037=CARTESIAN_POINT('Ctrl Pts',(-21.103794382086,-19.9244993534847,-7.38375626656748));
#63038=CARTESIAN_POINT('Ctrl Pts',(-21.1349820909847,-19.8401919830593,
-7.38824328403369));
#63039=CARTESIAN_POINT('Ctrl Pts',(-21.1660643193882,-19.7561697500644,
-7.39271512587973));
#63040=CARTESIAN_POINT('Ctrl Pts',(-21.1927730322953,-19.6704034844231,
-7.39718696772577));
#63041=CARTESIAN_POINT('Ctrl Pts',(-21.2149257129941,-19.5833537887784,
-7.40165880957181));
#63042=CARTESIAN_POINT('Ctrl Pts',(-21.2370311427379,-19.4964897673327,
-7.40612111312314));
#63043=CARTESIAN_POINT('Ctrl Pts',(-21.2545997969947,-19.4083481090824,
-7.41058341667445));
#63044=CARTESIAN_POINT('Ctrl Pts',(-21.2674980351242,-19.3194067310512,
-7.41504572022578));
#63045=CARTESIAN_POINT('Ctrl Pts',(-21.2803582069864,-19.2307278436205,
-7.41949485428542));
#63046=CARTESIAN_POINT('Ctrl Pts',(-21.2885753721633,-19.1412542906272,
-7.42394398834506));
#63047=CARTESIAN_POINT('Ctrl Pts',(-21.292066600817,-19.0514749505384,-7.4283931224047));
#63048=CARTESIAN_POINT('Ctrl Pts',(-21.2933474798422,-19.0185362676211,
-7.43002544244517));
#63049=CARTESIAN_POINT('Ctrl Pts',(-21.2939927168564,-18.9855565464178,
-7.43165776248564));
#63050=CARTESIAN_POINT('Ctrl Pts',(-21.2939999386838,-18.9525603024938,
-7.43329008252611));
#63051=CARTESIAN_POINT('Ctrl Pts',(-21.2898970146452,-18.9525588546298,
-7.4332901097715));
#63052=CARTESIAN_POINT('Ctrl Pts',(-21.288997505724,-18.4906083046144,-7.4561794192865));
#63053=CARTESIAN_POINT('Ctrl Pts',(-20.9482575273653,-17.1718695394144,
-7.52146066436198));
#63054=CARTESIAN_POINT('Ctrl Pts',(-19.0929371605554,-16.0796618992124,
-7.6158931522705));
#63055=CARTESIAN_POINT('Ctrl Pts',(-17.6442977293701,-16.5698109818192,
-7.68743633066402));
#63056=CARTESIAN_POINT('Ctrl Pts',(-17.175629477462,-16.9234129801345,-7.71658757349706));
#63057=CARTESIAN_POINT('',(-21.2941233546374,-18.9508698167174,-7.36670989022851));
#63058=CARTESIAN_POINT('Ctrl Pts',(-21.2976210191122,-18.9508682726504,
-7.36670989022851));
#63059=CARTESIAN_POINT('Ctrl Pts',(-21.2979707979485,-18.88753758729,-7.36987218932674));
#63060=CARTESIAN_POINT('Ctrl Pts',(-21.2671017039969,-17.9755793917529,
-7.41542642398544));
#63061=CARTESIAN_POINT('Ctrl Pts',(-20.1784866426459,-16.2917839998255,
-7.50337259420463));
#63062=CARTESIAN_POINT('Ctrl Pts',(-18.0960849448548,-16.2958827240454,
-7.5947114926735));
#63063=CARTESIAN_POINT('Ctrl Pts',(-17.2767521307163,-16.8392005158408,
-7.64365845558189));
#63064=CARTESIAN_POINT('Ctrl Pts',(-17.173230066991,-16.9202871232309,-7.65021348292981));
#63065=CARTESIAN_POINT('Ctrl Pts',(-17.1744641548914,-16.9218650419685,
-6.85004462002157));
#63066=CARTESIAN_POINT('Ctrl Pts',(-17.1078661424704,-16.9730251814325,
-6.85422899264962));
#63067=CARTESIAN_POINT('Ctrl Pts',(-17.0438780188053,-17.0273968013221,
-6.85841336527767));
#63068=CARTESIAN_POINT('Ctrl Pts',(-16.9828072236318,-17.0846693222688,
-6.86259773790572));
#63069=CARTESIAN_POINT('Ctrl Pts',(-16.9589890933644,-17.1070060932373,
-6.86422967886963));
#63070=CARTESIAN_POINT('Ctrl Pts',(-16.9356142875333,-17.1297837384485,
-6.86586161983354));
#63071=CARTESIAN_POINT('Ctrl Pts',(-16.9126993772538,-17.1529824788001,
-6.86749356079746));
#63072=CARTESIAN_POINT('Ctrl Pts',(-16.8539408046155,-17.2124688504872,
-6.8716781951905));
#63073=CARTESIAN_POINT('Ctrl Pts',(-16.7979903187279,-17.2749476638324,
-6.87586282958355));
#63074=CARTESIAN_POINT('Ctrl Pts',(-16.7451680193311,-17.3401230342645,
-6.8800474639766));
#63075=CARTESIAN_POINT('Ctrl Pts',(-16.6924209059394,-17.4052056356239,
-6.88422614206054));
#63076=CARTESIAN_POINT('Ctrl Pts',(-16.6427934219786,-17.4729768158299,
-6.88840482014449));
#63077=CARTESIAN_POINT('Ctrl Pts',(-16.5965688328438,-17.5431039762746,
-6.89258349822843));
#63078=CARTESIAN_POINT('Ctrl Pts',(-16.5495157011698,-17.6144881156707,
-6.89683707611387));
#63079=CARTESIAN_POINT('Ctrl Pts',(-16.5059889968457,-17.6883131849443,
-6.9010906539993));
#63080=CARTESIAN_POINT('Ctrl Pts',(-16.4662445138507,-17.7641931743589,
-6.90534423188474));
#63081=CARTESIAN_POINT('Ctrl Pts',(-16.4272705552134,-17.8386020821111,
-6.90951534586269));
#63082=CARTESIAN_POINT('Ctrl Pts',(-16.3919336983951,-17.9149865174728,
-6.91368645984064));
#63083=CARTESIAN_POINT('Ctrl Pts',(-16.3604304325482,-17.9929548975848,
-6.9178575738186));
#63084=CARTESIAN_POINT('Ctrl Pts',(-16.3289377379263,-18.0708971146538,
-6.92202728813897));
#63085=CARTESIAN_POINT('Ctrl Pts',(-16.3012762516654,-18.1504217947137,
-6.92619700245934));
#63086=CARTESIAN_POINT('Ctrl Pts',(-16.277594697511,-18.2311165212713,-6.93036671677971));
#63087=CARTESIAN_POINT('Ctrl Pts',(-16.253913986048,-18.3118083763642,-6.93453628272376));
#63088=CARTESIAN_POINT('Ctrl Pts',(-16.2342130538339,-18.3936697535165,
-6.9387058486678));
#63089=CARTESIAN_POINT('Ctrl Pts',(-16.2185906288469,-18.4762735076589,
-6.94287541461184));
#63090=CARTESIAN_POINT('Ctrl Pts',(-16.2024189386697,-18.5617815078941,
-6.94719157735077));
#63091=CARTESIAN_POINT('Ctrl Pts',(-16.190617990557,-18.6480845421363,-6.95150774008969));
#63092=CARTESIAN_POINT('Ctrl Pts',(-16.1832392059578,-18.7346998122939,
-6.95582390282861));
#63093=CARTESIAN_POINT('Ctrl Pts',(-16.1761007844907,-18.8184935991364,
-6.95999946702029));
#63094=CARTESIAN_POINT('Ctrl Pts',(-16.1731008165489,-18.9025791196894,
-6.96417503121196));
#63095=CARTESIAN_POINT('Ctrl Pts',(-16.1742327266829,-18.9865182046884,
-6.96835059540364));
#63096=CARTESIAN_POINT('Ctrl Pts',(-16.1754218069069,-19.0746968533245,
-6.97273705741619));
#63097=CARTESIAN_POINT('Ctrl Pts',(-16.1811710990057,-19.1627133020808,
-6.97712351942873));
#63098=CARTESIAN_POINT('Ctrl Pts',(-16.1914115149699,-19.2500667639851,
-6.98150998144128));
#63099=CARTESIAN_POINT('Ctrl Pts',(-16.2016519309342,-19.3374202258893,
-6.98589644345382));
#63100=CARTESIAN_POINT('Ctrl Pts',(-16.2163832985703,-19.4241101416678,
-6.99028290546636));
#63101=CARTESIAN_POINT('Ctrl Pts',(-16.2354754819719,-19.5096515334977,
-6.9946693674789));
#63102=CARTESIAN_POINT('Ctrl Pts',(-16.2536892057137,-19.5912570390867,
-6.99885400187195));
#63103=CARTESIAN_POINT('Ctrl Pts',(-16.2759390634244,-19.6721211400212,
-7.003038636265));
#63104=CARTESIAN_POINT('Ctrl Pts',(-16.3021495269225,-19.75181452637,-7.00722327065805));
#63105=CARTESIAN_POINT('Ctrl Pts',(-16.32832268307,-19.8313944790475,-7.01140194874199));
#63106=CARTESIAN_POINT('Ctrl Pts',(-16.3584451047931,-19.9098065938024,
-7.01558062682593));
#63107=CARTESIAN_POINT('Ctrl Pts',(-16.3923904554834,-19.9866326599468,
-7.01975930490988));
#63108=CARTESIAN_POINT('Ctrl Pts',(-16.4269442521886,-20.0648357781129,
-7.02401288279531));
#63109=CARTESIAN_POINT('Ctrl Pts',(-16.4654592728758,-20.1413949579938,
-7.02826646068075));
#63110=CARTESIAN_POINT('Ctrl Pts',(-16.5077494008733,-20.2158861775841,
-7.03252003856618));
#63111=CARTESIAN_POINT('Ctrl Pts',(-16.5492196522172,-20.288933239525,-7.03669115254414));
#63112=CARTESIAN_POINT('Ctrl Pts',(-16.5943197038782,-20.3599913900463,
-7.04086226652209));
#63113=CARTESIAN_POINT('Ctrl Pts',(-16.6428266524925,-20.428683456491,-7.04503338050004));
#63114=CARTESIAN_POINT('Ctrl Pts',(-16.6913173241317,-20.4973524726494,
-7.04920309482041));
#63115=CARTESIAN_POINT('Ctrl Pts',(-16.7432123571371,-20.5636566060813,
-7.05337280914078));
#63116=CARTESIAN_POINT('Ctrl Pts',(-16.7982454758471,-20.627247570427,-7.05754252346116));
#63117=CARTESIAN_POINT('Ctrl Pts',(-16.8532766362426,-20.6908362719333,
-7.0617120894052));
#63118=CARTESIAN_POINT('Ctrl Pts',(-16.9114453586341,-20.751711649014,-7.06588165534924));
#63119=CARTESIAN_POINT('Ctrl Pts',(-16.9724459211977,-20.8095594815388,
-7.07005122129329));
#63120=CARTESIAN_POINT('Ctrl Pts',(-17.0355911882886,-20.8694411724922,
-7.0743673840322));
#63121=CARTESIAN_POINT('Ctrl Pts',(-17.1017707529442,-20.9260780978832,
-7.07868354677113));
#63122=CARTESIAN_POINT('Ctrl Pts',(-17.1706064918292,-20.979165690961,-7.08299970951004));
#63123=CARTESIAN_POINT('Ctrl Pts',(-17.2371999137602,-21.030523961278,-7.08717527370172));
#63124=CARTESIAN_POINT('Ctrl Pts',(-17.3062787039752,-21.0785603570292,
-7.0913508378934));
#63125=CARTESIAN_POINT('Ctrl Pts',(-17.3774708722983,-21.1230432344145,
-7.09552640208508));
#63126=CARTESIAN_POINT('Ctrl Pts',(-17.4522587878001,-21.1697728361884,
-7.09991286409762));
#63127=CARTESIAN_POINT('Ctrl Pts',(-17.5293786750682,-21.2125802257264,
-7.10429932611016));
#63128=CARTESIAN_POINT('Ctrl Pts',(-17.6083720554812,-21.2512524286208,
-7.1086857881227));
#63129=CARTESIAN_POINT('Ctrl Pts',(-17.6873654358942,-21.2899246315151,
-7.11307225013524));
#63130=CARTESIAN_POINT('Ctrl Pts',(-17.7682317459862,-21.3244614898292,
-7.11745871214778));
#63131=CARTESIAN_POINT('Ctrl Pts',(-17.8504927560597,-21.3547099179687,
-7.12184517416032));
#63132=CARTESIAN_POINT('Ctrl Pts',(-17.9289688151197,-21.3835665710906,
-7.12602980855337));
#63133=CARTESIAN_POINT('Ctrl Pts',(-18.009006152961,-21.4086281659991,-7.13021444294641));
#63134=CARTESIAN_POINT('Ctrl Pts',(-18.0902029058993,-21.429725832619,-7.13439907733946));
#63135=CARTESIAN_POINT('Ctrl Pts',(-18.1712840853099,-21.4507934693218,
-7.1385777554234));
#63136=CARTESIAN_POINT('Ctrl Pts',(-18.2535209603944,-21.4679082701427,
-7.14275643350735));
#63137=CARTESIAN_POINT('Ctrl Pts',(-18.3364934985374,-21.4809500946628,
-7.14693511159129));
#63138=CARTESIAN_POINT('Ctrl Pts',(-18.4209532597953,-21.4942256845144,
-7.15118868947673));
#63139=CARTESIAN_POINT('Ctrl Pts',(-18.5061748645251,-21.5032806792605,
-7.15544226736216));
#63140=CARTESIAN_POINT('Ctrl Pts',(-18.5917010358989,-21.508042058499,-7.1596958452476));
#63141=CARTESIAN_POINT('Ctrl Pts',(-18.6755691155499,-21.5127111291099,
-7.16386695922555));
#63142=CARTESIAN_POINT('Ctrl Pts',(-18.7597295775162,-21.5132515520536,
-7.1680380732035));
#63143=CARTESIAN_POINT('Ctrl Pts',(-18.8437446259189,-21.5096465973785,
-7.17220918718146));
#63144=CARTESIAN_POINT('Ctrl Pts',(-18.9277314822607,-21.5060428523808,
-7.17637890150183));
#63145=CARTESIAN_POINT('Ctrl Pts',(-19.0115725627189,-21.4982965120596,
-7.1805486158222));
#63146=CARTESIAN_POINT('Ctrl Pts',(-19.0948308836175,-21.4864429513066,
-7.18471833014257));
#63147=CARTESIAN_POINT('Ctrl Pts',(-19.1780862418277,-21.4745898123542,
-7.18888789608662));
#63148=CARTESIAN_POINT('Ctrl Pts',(-19.2607584263887,-21.4586298092438,
-7.19305746203066));
#63149=CARTESIAN_POINT('Ctrl Pts',(-19.3424177464726,-21.4386499242509,
-7.19722702797471));
#63150=CARTESIAN_POINT('Ctrl Pts',(-19.426948107513,-21.4179675711496,-7.20154319071363));
#63151=CARTESIAN_POINT('Ctrl Pts',(-19.5103925419325,-21.3929775239273,
-7.20585935345255));
#63152=CARTESIAN_POINT('Ctrl Pts',(-19.5922902863025,-21.363832868264,-7.21017551619147));
#63153=CARTESIAN_POINT('Ctrl Pts',(-19.6715202202638,-21.3356375966935,
-7.21435108038315));
#63154=CARTESIAN_POINT('Ctrl Pts',(-19.7493022661266,-21.3035544560161,
-7.21852664457483));
#63155=CARTESIAN_POINT('Ctrl Pts',(-19.8252402968867,-21.2677708467054,
-7.22270220876651));
#63156=CARTESIAN_POINT('Ctrl Pts',(-19.9050137770549,-21.2301798923559,
-7.22708867077905));
#63157=CARTESIAN_POINT('Ctrl Pts',(-19.9827515495241,-21.1885050997007,
-7.23147513279159));
#63158=CARTESIAN_POINT('Ctrl Pts',(-20.058026370739,-21.1430166976971,-7.23586159480413));
#63159=CARTESIAN_POINT('Ctrl Pts',(-20.133301191954,-21.0975282956936,-7.24024805681667));
#63160=CARTESIAN_POINT('Ctrl Pts',(-20.2061126241217,-21.0482266726393,
-7.24463451882921));
#63161=CARTESIAN_POINT('Ctrl Pts',(-20.2760730898189,-20.9954310816997,
-7.24902098084176));
#63162=CARTESIAN_POINT('Ctrl Pts',(-20.3421228419793,-20.9455867065661,
-7.25316224442402));
#63163=CARTESIAN_POINT('Ctrl Pts',(-20.4058887674612,-20.892434299838,-7.25730350800628));
#63164=CARTESIAN_POINT('Ctrl Pts',(-20.4670153688586,-20.8362127616859,
-7.26144477158854));
#63165=CARTESIAN_POINT('Ctrl Pts',(-20.5280546973635,-20.7800714932714,
-7.26558012252323));
#63166=CARTESIAN_POINT('Ctrl Pts',(-20.5864618395735,-20.7208701082191,
-7.26971547345792));
#63167=CARTESIAN_POINT('Ctrl Pts',(-20.6419120481562,-20.6588894564384,
-7.27385082439262));
#63168=CARTESIAN_POINT('Ctrl Pts',(-20.6972986881794,-20.5969798597691,
-7.27798143452815));
#63169=CARTESIAN_POINT('Ctrl Pts',(-20.7497348173452,-20.5322976752762,
-7.28211204466369));
#63170=CARTESIAN_POINT('Ctrl Pts',(-20.7989315869957,-20.465161439182,-7.28624265479922));
#63171=CARTESIAN_POINT('Ctrl Pts',(-20.848098059321,-20.3980665482492,-7.29037072114094));
#63172=CARTESIAN_POINT('Ctrl Pts',(-20.8940288533086,-20.328520983131,-7.29449878748266));
#63173=CARTESIAN_POINT('Ctrl Pts',(-20.9364753744699,-20.2568763255013,
-7.29862685382437));
#63174=CARTESIAN_POINT('Ctrl Pts',(-20.9789091334294,-20.1852532089438,
-7.30275367899922));
#63175=CARTESIAN_POINT('Ctrl Pts',(-21.0178604599826,-20.11153265758,-7.30688050417406));
#63176=CARTESIAN_POINT('Ctrl Pts',(-21.0531249145872,-20.0360939214574,
-7.31100732934891));
#63177=CARTESIAN_POINT('Ctrl Pts',(-21.0883898804923,-19.9606540915461,
-7.31513421435873));
#63178=CARTESIAN_POINT('Ctrl Pts',(-21.1199676712092,-19.8834964546654,
-7.31926109936854));
#63179=CARTESIAN_POINT('Ctrl Pts',(-21.147701166054,-19.8050220870467,-7.32338798437836));
#63180=CARTESIAN_POINT('Ctrl Pts',(-21.175460263615,-19.7264752742866,-7.32751867920248));
#63181=CARTESIAN_POINT('Ctrl Pts',(-21.1993678247306,-19.6466097489538,
-7.3316493740266));
#63182=CARTESIAN_POINT('Ctrl Pts',(-21.2193162430201,-19.5658429540041,
-7.33578006885071));
#63183=CARTESIAN_POINT('Ctrl Pts',(-21.2392749611597,-19.4850344572076,
-7.33991289645233));
#63184=CARTESIAN_POINT('Ctrl Pts',(-21.2552703785522,-19.4033242264923,
-7.34404572405394));
#63185=CARTESIAN_POINT('Ctrl Pts',(-21.2672462583489,-19.3211387199431,
-7.34817855165556));
#63186=CARTESIAN_POINT('Ctrl Pts',(-21.2792406903518,-19.2388258972814,
-7.35231778154836));
#63187=CARTESIAN_POINT('Ctrl Pts',(-21.287203113202,-19.1560367972438,-7.35645701144116));
#63188=CARTESIAN_POINT('Ctrl Pts',(-21.291129302603,-19.0732011954116,-7.36059624133396));
#63189=CARTESIAN_POINT('Ctrl Pts',(-21.2930622985235,-19.0324184251309,
-7.36263412429881));
#63190=CARTESIAN_POINT('Ctrl Pts',(-21.2940177418851,-18.9916243590029,
-7.36467200726366));
#63191=CARTESIAN_POINT('Ctrl Pts',(-21.2939997505486,-18.9508698712832,
-7.36670989022851));
#63192=CARTESIAN_POINT('Origin',(-18.734,-18.952,1.76670989022851));
#63193=CARTESIAN_POINT('',(-17.1744641548914,-16.9218650419685,-6.05008448095771));
#63194=CARTESIAN_POINT('',(-17.1725993332886,-16.9194746534894,-6.11677129901302));
#63195=CARTESIAN_POINT('',(-17.1744641548914,-16.9218650419685,1.76670989022851));
#63196=CARTESIAN_POINT('',(-21.2939991231355,-18.954118854712,-6.6332901097715));
#63197=CARTESIAN_POINT('Ctrl Pts',(-17.1725993332886,-16.9194746534894,
-6.11677129901302));
#63198=CARTESIAN_POINT('Ctrl Pts',(-16.5753465810254,-17.3857070220397,
-6.1545808565094));
#63199=CARTESIAN_POINT('Ctrl Pts',(-15.7555915618427,-18.9714392322238,
-6.23478234956624));
#63200=CARTESIAN_POINT('Ctrl Pts',(-17.0342063769075,-21.4567939233708,
-6.35737577818358));
#63201=CARTESIAN_POINT('Ctrl Pts',(-19.9200692482785,-21.7370548823945,
-6.48455158486502));
#63202=CARTESIAN_POINT('Ctrl Pts',(-21.2201491927466,-20.0919179991473,
-6.57652302872766));
#63203=CARTESIAN_POINT('Ctrl Pts',(-21.2969228070761,-19.0983559330699,
-6.62610253702982));
#63204=CARTESIAN_POINT('Ctrl Pts',(-21.2956373923518,-18.9541202106712,
-6.6332901097715));
#63205=CARTESIAN_POINT('Ctrl Pts',(-21.2939991231355,-18.954118854712,-6.6332901097715));
#63206=CARTESIAN_POINT('Ctrl Pts',(-21.2940674480299,-18.8715687540988,
-6.63740642252224));
#63207=CARTESIAN_POINT('Ctrl Pts',(-21.2901386830331,-18.788875859184,-6.64152273527298));
#63208=CARTESIAN_POINT('Ctrl Pts',(-21.2821979940262,-18.7064659224447,
-6.64563904802373));
#63209=CARTESIAN_POINT('Ctrl Pts',(-21.2742662779566,-18.6241491085059,
-6.64975070936244));
#63210=CARTESIAN_POINT('Ctrl Pts',(-21.2623316869624,-18.5421150878493,
-6.65386237070115));
#63211=CARTESIAN_POINT('Ctrl Pts',(-21.2464314307689,-18.4607889397778,
-6.65797403203986));
#63212=CARTESIAN_POINT('Ctrl Pts',(-21.2305407999848,-18.3795120234587,
-6.66208320433541));
#63213=CARTESIAN_POINT('Ctrl Pts',(-21.2106893569247,-18.2989425946371,
-6.66619237663095));
#63214=CARTESIAN_POINT('Ctrl Pts',(-21.1869659077107,-18.2194986309849,
-6.6703015489265));
#63215=CARTESIAN_POINT('Ctrl Pts',(-21.1632492097462,-18.1400772755973,
-6.67440955182855));
#63216=CARTESIAN_POINT('Ctrl Pts',(-21.1356628286737,-18.0617812045221,
-6.67851755473059));
#63217=CARTESIAN_POINT('Ctrl Pts',(-21.1043458531986,-17.9850147176796,
-6.68262555763264));
#63218=CARTESIAN_POINT('Ctrl Pts',(-21.0730277445932,-17.9082454532244,
-6.686733709173));
#63219=CARTESIAN_POINT('Ctrl Pts',(-21.0379789552763,-17.8330063217982,
-6.69084186071337));
#63220=CARTESIAN_POINT('Ctrl Pts',(-20.9993866849094,-17.7596815996408,
-6.69495001225373));
#63221=CARTESIAN_POINT('Ctrl Pts',(-20.9607561733792,-17.6862842198592,
-6.69906223457025));
#63222=CARTESIAN_POINT('Ctrl Pts',(-20.9185753946451,-17.6148054564872,
-6.70317445688677));
#63223=CARTESIAN_POINT('Ctrl Pts',(-20.8730771242598,-17.5456042319217,
-6.70728667920329));
#63224=CARTESIAN_POINT('Ctrl Pts',(-20.8275541489319,-17.4763654320317,
-6.71140113440064));
#63225=CARTESIAN_POINT('Ctrl Pts',(-20.7787103793543,-17.4094070139061,
-6.715515589598));
#63226=CARTESIAN_POINT('Ctrl Pts',(-20.7268199445207,-17.3450561090317,
-6.71963004479535));
#63227=CARTESIAN_POINT('Ctrl Pts',(-20.6748438133914,-17.2805989295771,
-6.72375129495541));
#63228=CARTESIAN_POINT('Ctrl Pts',(-20.6198112918954,-17.2187582108668,
-6.72787254511546));
#63229=CARTESIAN_POINT('Ctrl Pts',(-20.5620341095491,-17.1598249822283,
-6.73199379527552));
#63230=CARTESIAN_POINT('Ctrl Pts',(-20.529745700387,-17.1268905239828,-6.73429692959298));
#63231=CARTESIAN_POINT('Ctrl Pts',(-20.4966007367167,-17.0948633881749,
-6.73660006391043));
#63232=CARTESIAN_POINT('Ctrl Pts',(-20.4626578964191,-17.0637887096122,
-6.73890319822789));
#63233=CARTESIAN_POINT('Ctrl Pts',(-20.400986123379,-17.0073281863674,-6.74308783262094));
#63234=CARTESIAN_POINT('Ctrl Pts',(-20.3364305466714,-16.9537872066972,
-6.74727246701399));
#63235=CARTESIAN_POINT('Ctrl Pts',(-20.2692989765721,-16.9034744198481,
-6.75145710140703));
#63236=CARTESIAN_POINT('Ctrl Pts',(-20.2022629599535,-16.8532332470235,
-6.75563577949098));
#63237=CARTESIAN_POINT('Ctrl Pts',(-20.1326585979522,-16.8062114135715,
-6.75981445757492));
#63238=CARTESIAN_POINT('Ctrl Pts',(-20.060828991676,-16.7626793686516,-6.76399313565886));
#63239=CARTESIAN_POINT('Ctrl Pts',(-19.9877118913304,-16.7183670431124,
-6.7682467135443));
#63240=CARTESIAN_POINT('Ctrl Pts',(-19.9122893426568,-16.6776711711576,
-6.77250029142973));
#63241=CARTESIAN_POINT('Ctrl Pts',(-19.8349567777298,-16.6408327248832,
-6.77675386931517));
#63242=CARTESIAN_POINT('Ctrl Pts',(-19.759123455476,-16.6047084637741,-6.78092498329312));
#63243=CARTESIAN_POINT('Ctrl Pts',(-19.6814539493098,-16.5722936025649,
-6.78509609727107));
#63244=CARTESIAN_POINT('Ctrl Pts',(-19.6023470115175,-16.5437696398416,
-6.78926721124902));
#63245=CARTESIAN_POINT('Ctrl Pts',(-19.5232666188221,-16.5152552486095,
-6.79343692556939));
#63246=CARTESIAN_POINT('Ctrl Pts',(-19.4427501848434,-16.4906293187767,
-6.79760663988977));
#63247=CARTESIAN_POINT('Ctrl Pts',(-19.3612154692014,-16.4700248278449,
-6.80177635421014));
#63248=CARTESIAN_POINT('Ctrl Pts',(-19.2796836549145,-16.4494210701093,
-6.80594592015419));
#63249=CARTESIAN_POINT('Ctrl Pts',(-19.1971340772291,-16.4328385786397,
-6.81011548609823));
#63250=CARTESIAN_POINT('Ctrl Pts',(-19.1139973178552,-16.4203598126071,
-6.81428505204228));
#63251=CARTESIAN_POINT('Ctrl Pts',(-19.027937572582,-16.407442308555,-6.8186012147812));
#63252=CARTESIAN_POINT('Ctrl Pts',(-18.941249108334,-16.3989225513938,-6.82291737752012));
#63253=CARTESIAN_POINT('Ctrl Pts',(-18.8544163259003,-16.3948336173693,
-6.82723354025904));
#63254=CARTESIAN_POINT('Ctrl Pts',(-18.7704121122212,-16.3908778799405,
-6.83140910445072));
#63255=CARTESIAN_POINT('Ctrl Pts',(-18.6862733092298,-16.3910686822566,
-6.8355846686424));
#63256=CARTESIAN_POINT('Ctrl Pts',(-18.6024375216843,-16.3953828377523,
-6.83976023283408));
#63257=CARTESIAN_POINT('Ctrl Pts',(-18.5143673878106,-16.3999148909862,
-6.84414669484662));
#63258=CARTESIAN_POINT('Ctrl Pts',(-18.4266322652434,-16.4089977253144,
-6.84853315685916));
#63259=CARTESIAN_POINT('Ctrl Pts',(-18.3397299608672,-16.4225433120446,
-6.8529196188717));
#63260=CARTESIAN_POINT('Ctrl Pts',(-18.252827656491,-16.4360888987749,-6.85730608088424));
#63261=CARTESIAN_POINT('Ctrl Pts',(-18.1667587226472,-16.4540970446291,
-6.86169254289678));
#63262=CARTESIAN_POINT('Ctrl Pts',(-18.0820028534405,-16.4764193164273,
-6.86607900490932));
#63263=CARTESIAN_POINT('Ctrl Pts',(-18.0004433963853,-16.4978997446872,
-6.87030003955252));
#63264=CARTESIAN_POINT('Ctrl Pts',(-17.9197934972278,-16.5234553456701,
-6.87452107419572));
#63265=CARTESIAN_POINT('Ctrl Pts',(-17.8404904722151,-16.5529917207818,
-6.87874210883892));
#63266=CARTESIAN_POINT('Ctrl Pts',(-17.7619934028019,-16.5822279181019,
-6.88292024516259));
#63267=CARTESIAN_POINT('Ctrl Pts',(-17.6848164097411,-16.6153642205991,
-6.88709838148626));
#63268=CARTESIAN_POINT('Ctrl Pts',(-17.6093723252539,-16.652258146401,-6.89127651780993));
#63269=CARTESIAN_POINT('Ctrl Pts',(-17.5327663263894,-16.6897202755698,
-6.89551900161289));
#63270=CARTESIAN_POINT('Ctrl Pts',(-17.4579475345501,-16.7310566404979,
-6.89976148541586));
#63271=CARTESIAN_POINT('Ctrl Pts',(-17.385329197042,-16.7760663922701,-6.90400396921883));
#63272=CARTESIAN_POINT('Ctrl Pts',(-17.3127108595338,-16.8210761440422,
-6.90824645302179));
#63273=CARTESIAN_POINT('Ctrl Pts',(-17.2422934238465,-16.8697590596227,
-6.91248893682476));
#63274=CARTESIAN_POINT('Ctrl Pts',(-17.1744641548914,-16.9218650419685,
-6.91673142062773));
#63275=CARTESIAN_POINT('',(-21.293999428374,-18.9502892327451,-6.5667098902584));
#63276=CARTESIAN_POINT('Ctrl Pts',(-21.293999428374,-18.9502892327451,-6.5667098902584));
#63277=CARTESIAN_POINT('Ctrl Pts',(-21.2939356382109,-18.8548333601135,
-6.57143929947811));
#63278=CARTESIAN_POINT('Ctrl Pts',(-21.2885288437516,-18.7595846663126,
-6.57616870869782));
#63279=CARTESIAN_POINT('Ctrl Pts',(-21.2778724975473,-18.6650980721178,
-6.58089811791753));
#63280=CARTESIAN_POINT('Ctrl Pts',(-21.2671635859909,-18.5701453968674,
-6.5856508562461));
#63281=CARTESIAN_POINT('Ctrl Pts',(-21.2511533349016,-18.4759625571734,
-6.59040359457466));
#63282=CARTESIAN_POINT('Ctrl Pts',(-21.2299860493113,-18.383094347327,-6.59515633290323));
#63283=CARTESIAN_POINT('Ctrl Pts',(-21.2086961910769,-18.2896883688573,
-6.59993659274375));
#63284=CARTESIAN_POINT('Ctrl Pts',(-21.1821895164639,-18.1976124823347,
-6.60471685258427));
#63285=CARTESIAN_POINT('Ctrl Pts',(-21.1506609174307,-18.1073994967067,
-6.60949711242479));
#63286=CARTESIAN_POINT('Ctrl Pts',(-21.1426476472041,-18.0844710744505,
-6.61071205742805));
#63287=CARTESIAN_POINT('Ctrl Pts',(-21.1343102131572,-18.061662873534,-6.61192700243132));
#63288=CARTESIAN_POINT('Ctrl Pts',(-21.1256522921827,-18.0389833992214,
-6.61314194743458));
#63289=CARTESIAN_POINT('Ctrl Pts',(-21.0958318198278,-17.9608684985716,
-6.61732658182763));
#63290=CARTESIAN_POINT('Ctrl Pts',(-21.062124806143,-17.8840707367778,-6.62151121622068));
#63291=CARTESIAN_POINT('Ctrl Pts',(-21.0246680532229,-17.8090039939071,
-6.62569585061373));
#63292=CARTESIAN_POINT('Ctrl Pts',(-20.9872646153543,-17.7340440992535,
-6.62987452869768));
#63293=CARTESIAN_POINT('Ctrl Pts',(-20.9461222434272,-17.6608107375728,
-6.63405320678162));
#63294=CARTESIAN_POINT('Ctrl Pts',(-20.9014264094921,-17.5896994606784,
-6.63823188486557));
#63295=CARTESIAN_POINT('Ctrl Pts',(-20.8559294348561,-17.5173135652524,
-6.64248546275101));
#63296=CARTESIAN_POINT('Ctrl Pts',(-20.8067505255347,-17.4471270300727,
-6.64673904063645));
#63297=CARTESIAN_POINT('Ctrl Pts',(-20.7541351457543,-17.3795325145211,
-6.65099261852188));
#63298=CARTESIAN_POINT('Ctrl Pts',(-20.7025398177813,-17.3132484505532,
-6.65516373249984));
#63299=CARTESIAN_POINT('Ctrl Pts',(-20.6476403712485,-17.2494571801025,
-6.65933484647779));
#63300=CARTESIAN_POINT('Ctrl Pts',(-20.5897118973504,-17.188499686977,-6.66350596045574));
#63301=CARTESIAN_POINT('Ctrl Pts',(-20.5318028619112,-17.127562648727,-6.66767567477611));
#63302=CARTESIAN_POINT('Ctrl Pts',(-20.4708671343697,-17.0694578324914,
-6.67184538909649));
#63303=CARTESIAN_POINT('Ctrl Pts',(-20.4072185463107,-17.0144913687206,
-6.67601510341686));
#63304=CARTESIAN_POINT('Ctrl Pts',(-20.3435722231415,-16.9595268608925,
-6.6801846693609));
#63305=CARTESIAN_POINT('Ctrl Pts',(-20.2772135801197,-16.9077007835214,
-6.68435423530495));
#63306=CARTESIAN_POINT('Ctrl Pts',(-20.2084905554454,-16.8592798558091,
-6.68852380124899));
#63307=CARTESIAN_POINT('Ctrl Pts',(-20.1373513140027,-16.8091565080122,
-6.69283996398791));
#63308=CARTESIAN_POINT('Ctrl Pts',(-20.0636787652557,-16.7626825189766,
-6.69715612672683));
#63309=CARTESIAN_POINT('Ctrl Pts',(-19.9878910926204,-16.7201045885062,
-6.70147228946575));
#63310=CARTESIAN_POINT('Ctrl Pts',(-19.9145721954497,-16.6789136296424,
-6.70564785365743));
#63311=CARTESIAN_POINT('Ctrl Pts',(-19.8392743011541,-16.6413689670526,
-6.70982341784911));
#63312=CARTESIAN_POINT('Ctrl Pts',(-19.7623989816003,-16.607646030429,-6.71399898204079));
#63313=CARTESIAN_POINT('Ctrl Pts',(-19.6816408724096,-16.5722198284451,
-6.71838544405333));
#63314=CARTESIAN_POINT('Ctrl Pts',(-19.5991423447411,-16.5410117758973,
-6.72277190606587));
#63315=CARTESIAN_POINT('Ctrl Pts',(-19.5153878511231,-16.5141663251737,
-6.72715836807841));
#63316=CARTESIAN_POINT('Ctrl Pts',(-19.4316333575051,-16.48732087445,-6.73154483009095));
#63317=CARTESIAN_POINT('Ctrl Pts',(-19.3466234783172,-16.4648381003647,
-6.73593129210349));
#63318=CARTESIAN_POINT('Ctrl Pts',(-19.2608535512399,-16.4468003401833,
-6.74031775411602));
#63319=CARTESIAN_POINT('Ctrl Pts',(-19.179022131781,-16.4295908639741,-6.74450279221877));
#63320=CARTESIAN_POINT('Ctrl Pts',(-19.0961943140763,-16.4163630651949,
-6.74868783032151));
#63321=CARTESIAN_POINT('Ctrl Pts',(-19.0127922770529,-16.4072259695101,
-6.75287286842426));
#63322=CARTESIAN_POINT('Ctrl Pts',(-18.9295335010323,-16.3981045687597,
-6.75705071782063));
#63323=CARTESIAN_POINT('Ctrl Pts',(-18.8457029204367,-16.3930599483569,
-6.761228567217));
#63324=CARTESIAN_POINT('Ctrl Pts',(-18.7617332667381,-16.3921502259086,
-6.76540641661338));
#63325=CARTESIAN_POINT('Ctrl Pts',(-18.6778456877694,-16.3912413926531,
-6.76958018244092));
#63326=CARTESIAN_POINT('Ctrl Pts',(-18.5938197628442,-16.3944594382541,
-6.77375394826846));
#63327=CARTESIAN_POINT('Ctrl Pts',(-18.5100929256538,-16.4018106693703,
-6.77792771409599));
#63328=CARTESIAN_POINT('Ctrl Pts',(-18.4264228070334,-16.409156920586,-6.78209865251434));
#63329=CARTESIAN_POINT('Ctrl Pts',(-18.3430518306328,-16.4206307562904,
-6.78626959093268));
#63330=CARTESIAN_POINT('Ctrl Pts',(-18.2604156415099,-16.4361864426406,
-6.79044052935102));
#63331=CARTESIAN_POINT('Ctrl Pts',(-18.1778106423856,-16.451736257691,-6.79460989350069));
#63332=CARTESIAN_POINT('Ctrl Pts',(-18.0959403308813,-16.4713647764078,
-6.79877925765036));
#63333=CARTESIAN_POINT('Ctrl Pts',(-18.0152320948012,-16.494974827468,-6.80294862180003));
#63334=CARTESIAN_POINT('Ctrl Pts',(-17.9344957178861,-16.5185931107307,
-6.8071194396971));
#63335=CARTESIAN_POINT('Ctrl Pts',(-17.8549226701269,-16.5461955784774,
-6.81129025759418));
#63336=CARTESIAN_POINT('Ctrl Pts',(-17.7769262676959,-16.5776348488631,
-6.81546107549126));
#63337=CARTESIAN_POINT('Ctrl Pts',(-17.6989179895211,-16.6090789061967,
-6.81963252843768));
#63338=CARTESIAN_POINT('Ctrl Pts',(-17.6224872570614,-16.644360746009,-6.82380398138411));
#63339=CARTESIAN_POINT('Ctrl Pts',(-17.5480265683097,-16.6832851613028,
-6.82797543433053));
#63340=CARTESIAN_POINT('Ctrl Pts',(-17.4734822892033,-16.722253273556,-6.83215157019405));
#63341=CARTESIAN_POINT('Ctrl Pts',(-17.4009128734863,-16.7648719041555,
-6.83632770605757));
#63342=CARTESIAN_POINT('Ctrl Pts',(-17.3306849630993,-16.8109005377591,
-6.84050384192108));
#63343=CARTESIAN_POINT('Ctrl Pts',(-17.2772041911319,-16.8459527961013,
-6.84368410128791));
#63344=CARTESIAN_POINT('Ctrl Pts',(-17.2250808115903,-16.8829816711023,
-6.84686436065474));
#63345=CARTESIAN_POINT('Ctrl Pts',(-17.1744641548914,-16.9218650419685,
-6.85004462002157));
#63346=CARTESIAN_POINT('Ctrl Pts',(-17.1744641548914,-16.9218650419685,
-6.05008448095771));
#63347=CARTESIAN_POINT('Ctrl Pts',(-17.1077757142765,-16.9730946477551,
-6.05425482184353));
#63348=CARTESIAN_POINT('Ctrl Pts',(-17.0436322004974,-17.027599857526,-6.05842516272933));
#63349=CARTESIAN_POINT('Ctrl Pts',(-16.9823602549826,-17.0850885924406,
-6.06259550361515));
#63350=CARTESIAN_POINT('Ctrl Pts',(-16.9210196771529,-17.1426417219966,
-6.06677051580929));
#63351=CARTESIAN_POINT('Ctrl Pts',(-16.8625574218519,-17.2031847300844,
-6.07094552800343));
#63352=CARTESIAN_POINT('Ctrl Pts',(-16.8072633052852,-17.2663886244928,
-6.07512054019757));
#63353=CARTESIAN_POINT('Ctrl Pts',(-16.7519329827071,-17.3296339041525,
-6.07929828614619));
#63354=CARTESIAN_POINT('Ctrl Pts',(-16.6997752124231,-17.3955431772239,
-6.08347603209481));
#63355=CARTESIAN_POINT('Ctrl Pts',(-16.651038064558,-17.4637562109992,-6.08765377804343));
#63356=CARTESIAN_POINT('Ctrl Pts',(-16.6022223342987,-17.5320792295344,
-6.09183826007106));
#63357=CARTESIAN_POINT('Ctrl Pts',(-16.5568384799099,-17.6027130346787,
-6.09602274209869));
#63358=CARTESIAN_POINT('Ctrl Pts',(-16.5150897345212,-17.6752708847399,
-6.10020722412632));
#63359=CARTESIAN_POINT('Ctrl Pts',(-16.5010171306903,-17.6997285748867,
-6.10161772298716));
#63360=CARTESIAN_POINT('Ctrl Pts',(-16.4873571552457,-17.7244046987976,
-6.103028221848));
#63361=CARTESIAN_POINT('Ctrl Pts',(-16.4741163568267,-17.7492839406919,
-6.10443872070885));
#63362=CARTESIAN_POINT('Ctrl Pts',(-16.4348338717473,-17.8230950824048,
-6.10862335510189));
#63363=CARTESIAN_POINT('Ctrl Pts',(-16.3990982578627,-17.8989701434485,
-6.11280798949494));
#63364=CARTESIAN_POINT('Ctrl Pts',(-16.3671315774458,-17.9765340240092,
-6.11699262388799));
#63365=CARTESIAN_POINT('Ctrl Pts',(-16.3352103976417,-18.0539875019864,
-6.12117130197193));
#63366=CARTESIAN_POINT('Ctrl Pts',(-16.3070476692934,-18.1331246030375,
-6.12534998005587));
#63367=CARTESIAN_POINT('Ctrl Pts',(-16.2828196558217,-18.2135455868409,
-6.12952865813981));
#63368=CARTESIAN_POINT('Ctrl Pts',(-16.2581573726209,-18.2954080589815,
-6.13378223602525));
#63369=CARTESIAN_POINT('Ctrl Pts',(-16.2375724777943,-18.3786004681759,
-6.13803581391068));
#63370=CARTESIAN_POINT('Ctrl Pts',(-16.2211996301978,-18.4626797556591,
-6.14228939179612));
#63371=CARTESIAN_POINT('Ctrl Pts',(-16.2051442022009,-18.5451290020872,
-6.14646050577408));
#63372=CARTESIAN_POINT('Ctrl Pts',(-16.1931390533222,-18.6284305735954,
-6.15063161975203));
#63373=CARTESIAN_POINT('Ctrl Pts',(-16.1852604222201,-18.7121530390888,
-6.15480273372998));
#63374=CARTESIAN_POINT('Ctrl Pts',(-16.1773844348688,-18.7958474107003,
-6.15897244805036));
#63375=CARTESIAN_POINT('Ctrl Pts',(-16.1736322583368,-18.8799619381736,
-6.16314216237074));
#63376=CARTESIAN_POINT('Ctrl Pts',(-16.1740284019004,-18.9640588939549,
-6.16731187669112));
#63377=CARTESIAN_POINT('Ctrl Pts',(-16.1744245313676,-19.0481528572053,
-6.17148144263516));
#63378=CARTESIAN_POINT('Ctrl Pts',(-16.1789686844146,-19.1322287899831,
-6.1756510085792));
#63379=CARTESIAN_POINT('Ctrl Pts',(-16.1876332505419,-19.2158491562505,
-6.17982057452324));
#63380=CARTESIAN_POINT('Ctrl Pts',(-16.1966024521253,-19.3024095114392,
-6.18413673726216));
#63381=CARTESIAN_POINT('Ctrl Pts',(-16.2099871509033,-19.3884811440156,
-6.18845290000108));
#63382=CARTESIAN_POINT('Ctrl Pts',(-16.2276984844482,-19.4735867263866,
-6.19276906274));
#63383=CARTESIAN_POINT('Ctrl Pts',(-16.2448328731658,-19.5559200033633,
-6.19694462693168));
#63384=CARTESIAN_POINT('Ctrl Pts',(-16.2660161808877,-19.6373487577949,
-6.20112019112336));
#63385=CARTESIAN_POINT('Ctrl Pts',(-16.2911167416148,-19.7174550188623,
-6.20529575531504));
#63386=CARTESIAN_POINT('Ctrl Pts',(-16.3174850719934,-19.8016072567417,
-6.20968221732758));
#63387=CARTESIAN_POINT('Ctrl Pts',(-16.3481765728435,-19.8842993445547,
-6.21406867934012));
#63388=CARTESIAN_POINT('Ctrl Pts',(-16.3829817631981,-19.9650711970168,
-6.21845514135267));
#63389=CARTESIAN_POINT('Ctrl Pts',(-16.4177869535527,-20.0458430494789,
-6.22284160336521));
#63390=CARTESIAN_POINT('Ctrl Pts',(-16.4567055084015,-20.1246941799628,
-6.22722806537775));
#63391=CARTESIAN_POINT('Ctrl Pts',(-16.4994739740983,-20.2011971179794,
-6.23161452739029));
#63392=CARTESIAN_POINT('Ctrl Pts',(-16.5402745992903,-20.2741800424133,
-6.23579916178334));
#63393=CARTESIAN_POINT('Ctrl Pts',(-16.5847305081231,-20.3452977698653,
-6.23998379617638));
#63394=CARTESIAN_POINT('Ctrl Pts',(-16.6326464991108,-20.4141605466913,
-6.24416843056943));
#63395=CARTESIAN_POINT('Ctrl Pts',(-16.680494287616,-20.4829253058779,-6.24834710865337));
#63396=CARTESIAN_POINT('Ctrl Pts',(-16.7317921151756,-20.5494411154154,
-6.2525257867373));
#63397=CARTESIAN_POINT('Ctrl Pts',(-16.786299271486,-20.6133433938069,-6.25670446482123));
#63398=CARTESIAN_POINT('Ctrl Pts',(-16.8417834293997,-20.678391074613,-6.26095804270667));
#63399=CARTESIAN_POINT('Ctrl Pts',(-16.9005928669018,-20.74073018676,-6.26521162059211));
#63400=CARTESIAN_POINT('Ctrl Pts',(-16.962427929971,-20.8000076841543,-6.26946519847754));
#63401=CARTESIAN_POINT('Ctrl Pts',(-17.0230641996815,-20.858135971591,-6.27363631245549));
#63402=CARTESIAN_POINT('Ctrl Pts',(-17.0866094791679,-20.91331996266,-6.27780742643344));
#63403=CARTESIAN_POINT('Ctrl Pts',(-17.1527422696948,-20.9652620272458,
-6.28197854041139));
#63404=CARTESIAN_POINT('Ctrl Pts',(-17.2188528687252,-21.0171866621702,
-6.28614825473177));
#63405=CARTESIAN_POINT('Ctrl Pts',(-17.2875488929265,-21.065871247202,-6.29031796905214));
#63406=CARTESIAN_POINT('Ctrl Pts',(-17.3584755491042,-21.1110582402955,
-6.29448768337252));
#63407=CARTESIAN_POINT('Ctrl Pts',(-17.429399681407,-21.1562436254418,-6.29865724931656));
#63408=CARTESIAN_POINT('Ctrl Pts',(-17.5025538994259,-21.1979314196434,
-6.30282681526059));
#63409=CARTESIAN_POINT('Ctrl Pts',(-17.5775553595551,-21.2359080090026,
-6.30699638120463));
#63410=CARTESIAN_POINT('Ctrl Pts',(-17.6551937784983,-21.2752198083945,
-6.31131254394355));
#63411=CARTESIAN_POINT('Ctrl Pts',(-17.7348112839516,-21.3105543371329,
-6.31562870668248));
#63412=CARTESIAN_POINT('Ctrl Pts',(-17.8159584194011,-21.3417279460833,
-6.3199448694214));
#63413=CARTESIAN_POINT('Ctrl Pts',(-17.8944621954484,-21.371886078001,-6.32412043361308));
#63414=CARTESIAN_POINT('Ctrl Pts',(-17.9743970142424,-21.3981501088934,
-6.32829599780477));
#63415=CARTESIAN_POINT('Ctrl Pts',(-18.0553401601613,-21.4204045093522,
-6.33247156199645));
#63416=CARTESIAN_POINT('Ctrl Pts',(-18.1403715519565,-21.4437829266733,
-6.336858024009));
#63417=CARTESIAN_POINT('Ctrl Pts',(-18.2265152388006,-21.4627358902474,
-6.34124448602154));
#63418=CARTESIAN_POINT('Ctrl Pts',(-18.3132709737048,-21.4771905049783,
-6.34563094803409));
#63419=CARTESIAN_POINT('Ctrl Pts',(-18.400026708609,-21.4916451197093,-6.35001741004663));
#63420=CARTESIAN_POINT('Ctrl Pts',(-18.487393906475,-21.5016013954773,-6.35440387205918));
#63421=CARTESIAN_POINT('Ctrl Pts',(-18.5748705298082,-21.5070494734381,
-6.35879033407172));
#63422=CARTESIAN_POINT('Ctrl Pts',(-18.6583222240302,-21.512246877256,-6.36297496846477));
#63423=CARTESIAN_POINT('Ctrl Pts',(-18.7421841184711,-21.5133611702432,
-6.36715960285781));
#63424=CARTESIAN_POINT('Ctrl Pts',(-18.826022833134,-21.5103455197025,-6.37134423725085));
#63425=CARTESIAN_POINT('Ctrl Pts',(-18.9097422137638,-21.5073341615672,
-6.37552291533479));
#63426=CARTESIAN_POINT('Ctrl Pts',(-18.9934380243477,-21.5002045527774,
-6.37970159341873));
#63427=CARTESIAN_POINT('Ctrl Pts',(-19.0766734176211,-21.4889617515556,
-6.38388027150267));
#63428=CARTESIAN_POINT('Ctrl Pts',(-19.1614007454988,-21.4775174312019,
-6.38813384938811));
#63429=CARTESIAN_POINT('Ctrl Pts',(-19.2456505065467,-21.4618109801084,
-6.39238742727355));
#63430=CARTESIAN_POINT('Ctrl Pts',(-19.3289636478325,-21.4419032627309,
-6.39664100515898));
#63431=CARTESIAN_POINT('Ctrl Pts',(-19.4106616013023,-21.4223814953014,
-6.40081211913693));
#63432=CARTESIAN_POINT('Ctrl Pts',(-19.4914584592899,-21.3988200192304,
-6.40498323311488));
#63433=CARTESIAN_POINT('Ctrl Pts',(-19.5709299408012,-21.3713280625394,
-6.40915434709283));
#63434=CARTESIAN_POINT('Ctrl Pts',(-19.6503747548895,-21.3438453310399,
-6.41332406141321));
#63435=CARTESIAN_POINT('Ctrl Pts',(-19.7284946413757,-21.3124348885696,
-6.41749377573358));
#63436=CARTESIAN_POINT('Ctrl Pts',(-19.8048810053292,-21.2772556574332,
-6.42166349005396));
#63437=CARTESIAN_POINT('Ctrl Pts',(-19.8812646511281,-21.2420776781249,
-6.425833055998));
#63438=CARTESIAN_POINT('Ctrl Pts',(-19.9559144795495,-21.2031313700067,
-6.43000262194205));
#63439=CARTESIAN_POINT('Ctrl Pts',(-20.0284436491279,-21.1606230188134,
-6.43417218788609));
#63440=CARTESIAN_POINT('Ctrl Pts',(-20.1035228548342,-21.116620126432,-6.43848835062502));
#63441=CARTESIAN_POINT('Ctrl Pts',(-20.1763290473291,-21.0688003143228,
-6.44280451336394));
#63442=CARTESIAN_POINT('Ctrl Pts',(-20.2464645244675,-21.0174420984931,
-6.44712067610286));
#63443=CARTESIAN_POINT('Ctrl Pts',(-20.314315345815,-20.967756871142,-6.45129624029455));
#63444=CARTESIAN_POINT('Ctrl Pts',(-20.3796664407519,-20.9147605602809,
-6.45547180448623));
#63445=CARTESIAN_POINT('Ctrl Pts',(-20.4421918593802,-20.8587460689739,
-6.45964736867791));
#63446=CARTESIAN_POINT('Ctrl Pts',(-20.5078752882633,-20.7999024188728,
-6.46403383069045));
#63447=CARTESIAN_POINT('Ctrl Pts',(-20.5704396751019,-20.7377280904822,
-6.46842029270299));
#63448=CARTESIAN_POINT('Ctrl Pts',(-20.6295529524493,-20.6726042556209,
-6.47280675471554));
#63449=CARTESIAN_POINT('Ctrl Pts',(-20.6886662297966,-20.6074804207597,
-6.47719321672808));
#63450=CARTESIAN_POINT('Ctrl Pts',(-20.7443280892575,-20.5394075767507,
-6.48157967874062));
#63451=CARTESIAN_POINT('Ctrl Pts',(-20.7962584977303,-20.4688025212726,
-6.48596614075316));
#63452=CARTESIAN_POINT('Ctrl Pts',(-20.8460908704135,-20.4010499743282,
-6.49017538570612));
#63453=CARTESIAN_POINT('Ctrl Pts',(-20.8926734978047,-20.3307132360494,
-6.49438463065908));
#63454=CARTESIAN_POINT('Ctrl Pts',(-20.9357293738869,-20.2581346654015,
-6.49859387561203));
#63455=CARTESIAN_POINT('Ctrl Pts',(-20.978722858141,-20.1856612676154,-6.50279702099133));
#63456=CARTESIAN_POINT('Ctrl Pts',(-21.0181995127225,-20.1109528753409,
-6.50700016637063));
#63457=CARTESIAN_POINT('Ctrl Pts',(-21.0539239335175,-20.0343829926107,
-6.51120331174993));
#63458=CARTESIAN_POINT('Ctrl Pts',(-21.0896068791139,-19.9579020056841,
-6.51540157737791));
#63459=CARTESIAN_POINT('Ctrl Pts',(-21.1215460556627,-19.8795642299174,
-6.51959984300589));
#63460=CARTESIAN_POINT('Ctrl Pts',(-21.1495512259748,-19.7997689984256,
-6.52379810863387));
#63461=CARTESIAN_POINT('Ctrl Pts',(-21.1775306085271,-19.7200472440895,
-6.52799250840908));
#63462=CARTESIAN_POINT('Ctrl Pts',(-21.2015830381501,-19.6388711282236,
-6.53218690818428));
#63463=CARTESIAN_POINT('Ctrl Pts',(-21.2215663308332,-19.556660028202,-6.53638130795949));
#63464=CARTESIAN_POINT('Ctrl Pts',(-21.2415389226779,-19.4744929513404,
-6.54057346167872));
#63465=CARTESIAN_POINT('Ctrl Pts',(-21.2574466025637,-19.391292431292,-6.54476561539796));
#63466=CARTESIAN_POINT('Ctrl Pts',(-21.2691973211301,-19.3074919730945,
-6.54895776911719));
#63467=CARTESIAN_POINT('Ctrl Pts',(-21.2809466969546,-19.2237010906845,
-6.55314944380356));
#63468=CARTESIAN_POINT('Ctrl Pts',(-21.288539988214,-19.1393108539585,-6.55734111848993));
#63469=CARTESIAN_POINT('Ctrl Pts',(-21.2919366299884,-19.0547628189733,
-6.5615327931763));
#63470=CARTESIAN_POINT('Ctrl Pts',(-21.2933350165072,-19.0199546642823,
-6.5632584921937));
#63471=CARTESIAN_POINT('Ctrl Pts',(-21.294022704555,-18.985119821685,-6.56498419121111));
#63472=CARTESIAN_POINT('Ctrl Pts',(-21.2939994283744,-18.9502892333484,
-6.56670989022851));
#63473=CARTESIAN_POINT('Origin',(-18.734,-18.952,1.76670989022851));
#63474=CARTESIAN_POINT('',(-17.1744641548914,-16.9218650419685,-5.25018234058848));
#63475=CARTESIAN_POINT('',(-17.1744641548914,-16.9218650419685,-5.31661774876036));
#63476=CARTESIAN_POINT('',(-17.1744641548914,-16.9218650419685,1.76670989022851));
#63477=CARTESIAN_POINT('',(-21.2939994369002,-18.9503020392335,-5.8332901097715));
#63478=CARTESIAN_POINT('Ctrl Pts',(-17.1744641548914,-16.9218650419685,
-5.31661774876036));
#63479=CARTESIAN_POINT('Ctrl Pts',(-17.1078003775552,-16.9730757015923,
-5.3208013195428));
#63480=CARTESIAN_POINT('Ctrl Pts',(-17.0437399774918,-17.0275131658057,
-5.32498489032524));
#63481=CARTESIAN_POINT('Ctrl Pts',(-16.9825941690676,-17.084869148834,-5.32916846110767));
#63482=CARTESIAN_POINT('Ctrl Pts',(-16.929973447652,-17.1342284308883,-5.33276874898248));
#63483=CARTESIAN_POINT('Ctrl Pts',(-16.8795107690236,-17.1857484040204,
-5.33636903685729));
#63484=CARTESIAN_POINT('Ctrl Pts',(-16.8313804354228,-17.239213150305,-5.3399693247321));
#63485=CARTESIAN_POINT('Ctrl Pts',(-16.7754382840342,-17.3013555188872,
-5.34415395912515));
#63486=CARTESIAN_POINT('Ctrl Pts',(-16.7224397206528,-17.3663571440022,
-5.3483385935182));
#63487=CARTESIAN_POINT('Ctrl Pts',(-16.6726908063355,-17.4339076417707,
-5.35252322791125));
#63488=CARTESIAN_POINT('Ctrl Pts',(-16.62301270344,-17.5013619897668,-5.35670190599519));
#63489=CARTESIAN_POINT('Ctrl Pts',(-16.5765753324319,-17.5713576368076,
-5.36088058407914));
#63490=CARTESIAN_POINT('Ctrl Pts',(-16.533646260122,-17.6435492292773,-5.36505926216308));
#63491=CARTESIAN_POINT('Ctrl Pts',(-16.4899477150434,-17.7170348041589,
-5.36931284004852));
#63492=CARTESIAN_POINT('Ctrl Pts',(-16.4498848008427,-17.7927954651138,
-5.37356641793395));
#63493=CARTESIAN_POINT('Ctrl Pts',(-16.4136951701205,-17.8704337762127,
-5.37781999581939));
#63494=CARTESIAN_POINT('Ctrl Pts',(-16.378207146008,-17.9465669171522,-5.38199110979734));
#63495=CARTESIAN_POINT('Ctrl Pts',(-16.3464437665668,-18.0245051179384,
-5.38616222377529));
#63496=CARTESIAN_POINT('Ctrl Pts',(-16.3185831851716,-18.1038481205325,
-5.39033333775324));
#63497=CARTESIAN_POINT('Ctrl Pts',(-16.2907319526636,-18.1831644988157,
-5.39450305207362));
#63498=CARTESIAN_POINT('Ctrl Pts',(-16.2667810695588,-18.2638843090192,
-5.39867276639399));
#63499=CARTESIAN_POINT('Ctrl Pts',(-16.2468600106956,-18.3455886927152,
-5.40284248071436));
#63500=CARTESIAN_POINT('Ctrl Pts',(-16.2269396607091,-18.4272901690186,
-5.40701204665841));
#63501=CARTESIAN_POINT('Ctrl Pts',(-16.2110489579957,-18.5099757020134,
-5.41118161260245));
#63502=CARTESIAN_POINT('Ctrl Pts',(-16.1992667534716,-18.5932140346339,
-5.4153511785465));
#63503=CARTESIAN_POINT('Ctrl Pts',(-16.1870703011713,-18.6793789243438,
-5.41966734128542));
#63504=CARTESIAN_POINT('Ctrl Pts',(-16.1792767060087,-18.7661356875971,
-5.42398350402433));
#63505=CARTESIAN_POINT('Ctrl Pts',(-16.1759149870658,-18.8529996636308,
-5.42829966676326));
#63506=CARTESIAN_POINT('Ctrl Pts',(-16.1726627757638,-18.9370340547817,
-5.43247523095494));
#63507=CARTESIAN_POINT('Ctrl Pts',(-16.1735580857934,-19.0211683105536,
-5.43665079514662));
#63508=CARTESIAN_POINT('Ctrl Pts',(-16.1785740672325,-19.1049650356758,
-5.4408263593383));
#63509=CARTESIAN_POINT('Ctrl Pts',(-16.1838433939698,-19.1929941341762,
-5.44521282135084));
#63510=CARTESIAN_POINT('Ctrl Pts',(-16.1936605371381,-19.2806501283314,
-5.44959928336338));
#63511=CARTESIAN_POINT('Ctrl Pts',(-16.2079333028748,-19.3674359657935,
-5.45398574537592));
#63512=CARTESIAN_POINT('Ctrl Pts',(-16.2222060686114,-19.4542218032555,
-5.45837220738846));
#63513=CARTESIAN_POINT('Ctrl Pts',(-16.2409342590202,-19.5401369333207,
-5.462758669401));
#63514=CARTESIAN_POINT('Ctrl Pts',(-16.2639654295305,-19.6247029215675,
-5.46714513141354));
#63515=CARTESIAN_POINT('Ctrl Pts',(-16.2859369017452,-19.7053779033382,
-5.47132976580659));
#63516=CARTESIAN_POINT('Ctrl Pts',(-16.3119058645756,-19.7851254547589,
-5.47551440019964));
#63517=CARTESIAN_POINT('Ctrl Pts',(-16.3417769993438,-19.863520222009,-5.47969903459269));
#63518=CARTESIAN_POINT('Ctrl Pts',(-16.3716056162489,-19.9418034040112,
-5.48387771267663));
#63519=CARTESIAN_POINT('Ctrl Pts',(-16.4053252101866,-20.0187372003264,
-5.48805639076057));
#63520=CARTESIAN_POINT('Ctrl Pts',(-16.4427902222593,-20.0939096962481,
-5.49223506884451));
#63521=CARTESIAN_POINT('Ctrl Pts',(-16.4809267677478,-20.1704296051337,
-5.49648864672995));
#63522=CARTESIAN_POINT('Ctrl Pts',(-16.5229441986227,-20.2451239847432,
-5.50074222461539));
#63523=CARTESIAN_POINT('Ctrl Pts',(-16.5686369710085,-20.3175778823182,
-5.50499580250082));
#63524=CARTESIAN_POINT('Ctrl Pts',(-16.6134438998394,-20.3886271197065,
-5.50916691647877));
#63525=CARTESIAN_POINT('Ctrl Pts',(-16.6617846778615,-20.4575215650235,
-5.51333803045673));
#63526=CARTESIAN_POINT('Ctrl Pts',(-16.7134191824493,-20.5238947673893,
-5.51750914443468));
#63527=CARTESIAN_POINT('Ctrl Pts',(-16.7650363605803,-20.5902456975861,
-5.52167885875505));
#63528=CARTESIAN_POINT('Ctrl Pts',(-16.8199447880143,-20.6540767022587,
-5.52584857307543));
#63529=CARTESIAN_POINT('Ctrl Pts',(-16.8778623533737,-20.7150521934352,
-5.5300182873958));
#63530=CARTESIAN_POINT('Ctrl Pts',(-16.9357778577776,-20.776025514842,-5.53418785333984));
#63531=CARTESIAN_POINT('Ctrl Pts',(-16.9967019697692,-20.8341431918207,
-5.53835741928388));
#63532=CARTESIAN_POINT('Ctrl Pts',(-17.0603147509096,-20.8891054919589,
-5.54252698522793));
#63533=CARTESIAN_POINT('Ctrl Pts',(-17.12616407896,-20.9460001987665,-5.54684314796685));
#63534=CARTESIAN_POINT('Ctrl Pts',(-17.1948942620563,-20.999513169412,-5.55115931070577));
#63535=CARTESIAN_POINT('Ctrl Pts',(-17.2661134846746,-21.0493576657609,
-5.55547547344469));
#63536=CARTESIAN_POINT('Ctrl Pts',(-17.3350127486071,-21.097578482884,-5.55965103763637));
#63537=CARTESIAN_POINT('Ctrl Pts',(-17.4062409575147,-21.1423659457519,
-5.56382660182805));
#63538=CARTESIAN_POINT('Ctrl Pts',(-17.4794157978407,-21.183505877136,-5.56800216601973));
#63539=CARTESIAN_POINT('Ctrl Pts',(-17.5562865253949,-21.2267236886533,
-5.57238862803227));
#63540=CARTESIAN_POINT('Ctrl Pts',(-17.6353051780177,-21.2659155519541,
-5.57677509004481));
#63541=CARTESIAN_POINT('Ctrl Pts',(-17.7160039105556,-21.3008899424784,
-5.58116155205735));
#63542=CARTESIAN_POINT('Ctrl Pts',(-17.7967026430936,-21.3358643330026,
-5.5855480140699));
#63543=CARTESIAN_POINT('Ctrl Pts',(-17.8790808853744,-21.3666211190642,
-5.58993447608243));
#63544=CARTESIAN_POINT('Ctrl Pts',(-17.9626538344086,-21.393029514944,-5.59432093809497));
#63545=CARTESIAN_POINT('Ctrl Pts',(-18.042381468173,-21.4182228213826,-5.59850557248802));
#63546=CARTESIAN_POINT('Ctrl Pts',(-18.123493045634,-21.4395528703718,-5.60269020688107));
#63547=CARTESIAN_POINT('Ctrl Pts',(-18.2055793173495,-21.4568695738795,
-5.60687484127412));
#63548=CARTESIAN_POINT('Ctrl Pts',(-18.2875487494174,-21.474161629203,-5.61105351935806));
#63549=CARTESIAN_POINT('Ctrl Pts',(-18.370489673737,-21.4874515917234,-5.615232197442));
#63550=CARTESIAN_POINT('Ctrl Pts',(-18.4539769469565,-21.4966388918203,
-5.61941087552594));
#63551=CARTESIAN_POINT('Ctrl Pts',(-18.5389606695472,-21.5059908676685,
-5.62366445341137));
#63552=CARTESIAN_POINT('Ctrl Pts',(-18.624510060566,-21.511091508697,-5.62791803129681));
#63553=CARTESIAN_POINT('Ctrl Pts',(-18.7101649534091,-21.5118890387191,
-5.63217160918224));
#63554=CARTESIAN_POINT('Ctrl Pts',(-18.7941592590127,-21.5126711070654,
-5.63634272316019));
#63555=CARTESIAN_POINT('Ctrl Pts',(-18.87825453103,-21.5093154194064,-5.64051383713815));
#63556=CARTESIAN_POINT('Ctrl Pts',(-18.9620126684401,-21.5018255279589,
-5.6446849511161));
#63557=CARTESIAN_POINT('Ctrl Pts',(-19.0457426999984,-21.4943381498168,
-5.64885466543647));
#63558=CARTESIAN_POINT('Ctrl Pts',(-19.1291353638018,-21.4827193639704,
-5.65302437975684));
#63559=CARTESIAN_POINT('Ctrl Pts',(-19.2117557819361,-21.4670247340387,
-5.65719409407722));
#63560=CARTESIAN_POINT('Ctrl Pts',(-19.2943732600814,-21.4513306625894,
-5.66136366002126));
#63561=CARTESIAN_POINT('Ctrl Pts',(-19.3762180954026,-21.4315611221138,
-5.66553322596531));
#63562=CARTESIAN_POINT('Ctrl Pts',(-19.4568650837657,-21.4078228907379,
-5.66970279190935));
#63563=CARTESIAN_POINT('Ctrl Pts',(-19.5403475207508,-21.3832500524311,
-5.67401895464827));
#63564=CARTESIAN_POINT('Ctrl Pts',(-19.6225458049915,-21.3544244012911,
-5.67833511738719));
#63565=CARTESIAN_POINT('Ctrl Pts',(-19.7030067527822,-21.3215201862534,
-5.68265128012611));
#63566=CARTESIAN_POINT('Ctrl Pts',(-19.7808466936617,-21.2896878225597,
-5.68682684431779));
#63567=CARTESIAN_POINT('Ctrl Pts',(-19.8570603406958,-21.2540387751659,
-5.69100240850947));
#63568=CARTESIAN_POINT('Ctrl Pts',(-19.9312606656523,-21.214778579199,-5.69517797270115));
#63569=CARTESIAN_POINT('Ctrl Pts',(-20.0092086726279,-21.173535444066,-5.69956443471369));
#63570=CARTESIAN_POINT('Ctrl Pts',(-20.0849341253745,-21.1283070744553,
-5.70395089672623));
#63571=CARTESIAN_POINT('Ctrl Pts',(-20.1580227463384,-21.0793831854912,
-5.70833735873878));
#63572=CARTESIAN_POINT('Ctrl Pts',(-20.2311113673023,-21.0304592965271,
-5.71272382075132));
#63573=CARTESIAN_POINT('Ctrl Pts',(-20.3015627371329,-20.977840296355,-5.71711028276386));
#63574=CARTESIAN_POINT('Ctrl Pts',(-20.3690044710744,-20.9218630357379,
-5.72149674477641));
#63575=CARTESIAN_POINT('Ctrl Pts',(-20.4324580482223,-20.8691959820087,
-5.72562381401755));
#63576=CARTESIAN_POINT('Ctrl Pts',(-20.493497997814,-20.8133485129555,-5.72975088325869));
#63577=CARTESIAN_POINT('Ctrl Pts',(-20.5517814829091,-20.7545732940418,
-5.73387795249983));
#63578=CARTESIAN_POINT('Ctrl Pts',(-20.6102782700971,-20.6955829734199,
-5.73802012571948));
#63579=CARTESIAN_POINT('Ctrl Pts',(-20.6659979620833,-20.6336436795686,
-5.74216229893913));
#63580=CARTESIAN_POINT('Ctrl Pts',(-20.7186255971236,-20.5690532580103,
-5.74630447215879));
#63581=CARTESIAN_POINT('Ctrl Pts',(-20.7709257203661,-20.5048647949491,
-5.75042086784546));
#63582=CARTESIAN_POINT('Ctrl Pts',(-20.8201718394842,-20.4380584608902,
-5.75453726353214));
#63583=CARTESIAN_POINT('Ctrl Pts',(-20.8660914253506,-20.368963709467,-5.75865365921881));
#63584=CARTESIAN_POINT('Ctrl Pts',(-20.9119829684086,-20.299911153783,-5.76276754104798));
#63585=CARTESIAN_POINT('Ctrl Pts',(-20.9545517475122,-20.228573347296,-5.76688142287715));
#63586=CARTESIAN_POINT('Ctrl Pts',(-20.993566969393,-20.1553108953334,-5.77099530470633));
#63587=CARTESIAN_POINT('Ctrl Pts',(-21.0325708263852,-20.0820697842621,
-5.77510798818761));
#63588=CARTESIAN_POINT('Ctrl Pts',(-21.0680229592545,-20.006905559054,-5.7792206716689));
#63589=CARTESIAN_POINT('Ctrl Pts',(-21.0997379788823,-19.9302043831808,
-5.78333335515018));
#63590=CARTESIAN_POINT('Ctrl Pts',(-21.1318415000294,-19.8525636359715,
-5.78749641803529));
#63591=CARTESIAN_POINT('Ctrl Pts',(-21.1601155043872,-19.7733484709675,
-5.7916594809204));
#63592=CARTESIAN_POINT('Ctrl Pts',(-21.1844181339265,-19.6929797358392,
-5.79582254380551));
#63593=CARTESIAN_POINT('Ctrl Pts',(-21.2084475698834,-19.6135144512045,
-5.79993880837766));
#63594=CARTESIAN_POINT('Ctrl Pts',(-21.2285944016387,-19.5329218806182,
-5.80405507294981));
#63595=CARTESIAN_POINT('Ctrl Pts',(-21.2447724368935,-19.45162162697,-5.80817133752195));
#63596=CARTESIAN_POINT('Ctrl Pts',(-21.2612263672263,-19.3689349046021,
-5.81235779956354));
#63597=CARTESIAN_POINT('Ctrl Pts',(-21.2735747867911,-19.2855166404038,
-5.81654426160514));
#63598=CARTESIAN_POINT('Ctrl Pts',(-21.281781944964,-19.2018142528271,-5.82073072364673));
#63599=CARTESIAN_POINT('Ctrl Pts',(-21.2899891031369,-19.1181118652504,
-5.82491718568832));
#63600=CARTESIAN_POINT('Ctrl Pts',(-21.2940550344004,-19.0341258661346,
-5.82910364772991));
#63601=CARTESIAN_POINT('Ctrl Pts',(-21.2939994369002,-18.9503020392335,
-5.8332901097715));
#63602=CARTESIAN_POINT('Ctrl Pts',(-21.2967673690372,-18.950300203358,-5.8332901097715));
#63603=CARTESIAN_POINT('Ctrl Pts',(-21.2975539709192,-18.8475231740461,
-5.83841759033362));
#63604=CARTESIAN_POINT('Ctrl Pts',(-21.2452320420947,-17.8958349639979,
-5.88593700645621));
#63605=CARTESIAN_POINT('Ctrl Pts',(-20.0538051353946,-16.2277743551153,
-5.97584835813928));
#63606=CARTESIAN_POINT('Ctrl Pts',(-18.0187464898779,-16.3260865960557,
-6.06521460732434));
#63607=CARTESIAN_POINT('Ctrl Pts',(-17.2449841505655,-16.8629690205255,
-6.11218892094892));
#63608=CARTESIAN_POINT('Ctrl Pts',(-17.1725993332886,-16.9194746534894,
-6.11677129901302));
#63609=CARTESIAN_POINT('',(-21.2939992944986,-18.9539005700933,-5.76670989019962));
#63610=CARTESIAN_POINT('Ctrl Pts',(-21.293999294499,-18.9539005695104,-5.76670989022851));
#63611=CARTESIAN_POINT('Ctrl Pts',(-21.2940618231948,-18.8696766480678,
-5.77088500205647));
#63612=CARTESIAN_POINT('Ctrl Pts',(-21.2899635861128,-18.7854119279347,
-5.77506011388444));
#63613=CARTESIAN_POINT('Ctrl Pts',(-21.2817191504239,-18.7015461508316,
-5.7792352257124));
#63614=CARTESIAN_POINT('Ctrl Pts',(-21.2734754980237,-18.6176883416611,
-5.78340994087069));
#63615=CARTESIAN_POINT('Ctrl Pts',(-21.2610864747303,-18.5342298557722,
-5.78758465602898));
#63616=CARTESIAN_POINT('Ctrl Pts',(-21.2446185572459,-18.4516056954637,
-5.79175937118727));
#63617=CARTESIAN_POINT('Ctrl Pts',(-21.2281473245846,-18.3689649019827,
-5.79593492676267));
#63618=CARTESIAN_POINT('Ctrl Pts',(-21.2075956572652,-18.2871592164316,
-5.80011048233806));
#63619=CARTESIAN_POINT('Ctrl Pts',(-21.1830809475489,-18.2066125085882,
-5.80428603791345));
#63620=CARTESIAN_POINT('Ctrl Pts',(-21.1585369190254,-18.1259694694636,
-5.8084665873195));
#63621=CARTESIAN_POINT('Ctrl Pts',(-21.1300205198882,-18.0465888526481,
-5.81264713672554));
#63622=CARTESIAN_POINT('Ctrl Pts',(-21.0976986239761,-17.9688780263805,
-5.81682768613158));
#63623=CARTESIAN_POINT('Ctrl Pts',(-21.065355928357,-17.8911171918331,-5.8210109257945));
#63624=CARTESIAN_POINT('Ctrl Pts',(-21.0292030575735,-17.8150287001824,
-5.82519416545742));
#63625=CARTESIAN_POINT('Ctrl Pts',(-20.9894534545794,-17.740996402059,-5.82937740512034));
#63626=CARTESIAN_POINT('Ctrl Pts',(-20.949632004209,-17.6668302906149,-5.83356820598567));
#63627=CARTESIAN_POINT('Ctrl Pts',(-20.9062010761476,-17.5947281861657,
-5.83775900685099));
#63628=CARTESIAN_POINT('Ctrl Pts',(-20.859418003607,-17.5250457926257,-5.84194980771632));
#63629=CARTESIAN_POINT('Ctrl Pts',(-20.8291383592866,-17.4799449051208,
-5.84466224092621));
#63630=CARTESIAN_POINT('Ctrl Pts',(-20.7974553185201,-17.435857034571,-5.84737467413609));
#63631=CARTESIAN_POINT('Ctrl Pts',(-20.7644472985012,-17.392870830236,-5.85008710734598));
#63632=CARTESIAN_POINT('Ctrl Pts',(-20.7135238341689,-17.3265534188316,
-5.85427174173903));
#63633=CARTESIAN_POINT('Ctrl Pts',(-20.6592531496868,-17.262610070515,-5.85845637613208));
#63634=CARTESIAN_POINT('Ctrl Pts',(-20.6018847443059,-17.2013982228989,
-5.86264101052513));
#63635=CARTESIAN_POINT('Ctrl Pts',(-20.5445979957492,-17.1402735027715,
-5.86681968860907));
#63636=CARTESIAN_POINT('Ctrl Pts',(-20.4842225962896,-17.0818728934348,
-5.87099836669301));
#63637=CARTESIAN_POINT('Ctrl Pts',(-20.4210494366143,-17.0265223453856,
-5.87517704477696));
#63638=CARTESIAN_POINT('Ctrl Pts',(-20.3567439434536,-16.9701796785424,
-5.87943062266239));
#63639=CARTESIAN_POINT('Ctrl Pts',(-20.2895396974698,-16.9169978755988,
-5.88368420054783));
#63640=CARTESIAN_POINT('Ctrl Pts',(-20.2197842460677,-16.867282951061,-5.88793777843326));
#63641=CARTESIAN_POINT('Ctrl Pts',(-20.1513811402077,-16.8185318473461,
-5.89210889241121));
#63642=CARTESIAN_POINT('Ctrl Pts',(-20.0805252582504,-16.7731146765031,
-5.89628000638917));
#63643=CARTESIAN_POINT('Ctrl Pts',(-20.0075777510545,-16.7312794610715,
-5.90045112036712));
#63644=CARTESIAN_POINT('Ctrl Pts',(-19.9346547220991,-16.6894582838504,
-5.90462083468749));
#63645=CARTESIAN_POINT('Ctrl Pts',(-19.8596418605523,-16.6512169036013,
-5.90879054900787));
#63646=CARTESIAN_POINT('Ctrl Pts',(-19.7829274662086,-16.6167588624227,
-5.91296026332824));
#63647=CARTESIAN_POINT('Ctrl Pts',(-19.7062158016923,-16.5823020474091,
-5.91712982927229));
#63648=CARTESIAN_POINT('Ctrl Pts',(-19.6278031447566,-16.5516284915072,
-5.92129939521634));
#63649=CARTESIAN_POINT('Ctrl Pts',(-19.5480992,-16.5248942147983,-5.92546896116038));
#63650=CARTESIAN_POINT('Ctrl Pts',(-19.4655929628713,-16.4972199939008,
-5.9297851238993));
#63651=CARTESIAN_POINT('Ctrl Pts',(-19.3817034451241,-16.4737673840696,
-5.93410128663822));
#63652=CARTESIAN_POINT('Ctrl Pts',(-19.2969019322694,-16.4546531248848,
-5.93841744937714));
#63653=CARTESIAN_POINT('Ctrl Pts',(-19.2148628197763,-16.4361615106825,
-5.94259301356882));
#63654=CARTESIAN_POINT('Ctrl Pts',(-19.1319706883696,-16.4217299783601,
-5.9467685777605));
#63655=CARTESIAN_POINT('Ctrl Pts',(-19.0486605152115,-16.411411729507,-5.95094414195218));
#63656=CARTESIAN_POINT('Ctrl Pts',(-18.9611425432584,-16.4005723304336,
-5.95533060396472));
#63657=CARTESIAN_POINT('Ctrl Pts',(-18.8731637715279,-16.3942727005953,
-5.95971706597726));
#63658=CARTESIAN_POINT('Ctrl Pts',(-18.7852297301449,-16.3925126461048,
-5.9641035279898));
#63659=CARTESIAN_POINT('Ctrl Pts',(-18.6972956887618,-16.3907525916143,
-5.96848999000234));
#63660=CARTESIAN_POINT('Ctrl Pts',(-18.609406955249,-16.3935320181048,-5.97287645201488));
#63661=CARTESIAN_POINT('Ctrl Pts',(-18.5220617179687,-16.4007880988421,
-5.97726291402742));
#63662=CARTESIAN_POINT('Ctrl Pts',(-18.4387429644685,-16.4077096851948,
-5.98144716675304));
#63663=CARTESIAN_POINT('Ctrl Pts',(-18.3556086019078,-16.4187300407395,
-5.98563141947867));
#63664=CARTESIAN_POINT('Ctrl Pts',(-18.273094108763,-16.4338328571314,-5.98981567220429));
#63665=CARTESIAN_POINT('Ctrl Pts',(-18.190691343874,-16.4489152236451,-5.99399425926754));
#63666=CARTESIAN_POINT('Ctrl Pts',(-18.1089072302701,-16.4680689925798,
-5.99817284633079));
#63667=CARTESIAN_POINT('Ctrl Pts',(-18.0281732667358,-16.4912260114733,
-6.00235143339404));
#63668=CARTESIAN_POINT('Ctrl Pts',(-17.9475320674901,-16.5143564226754,
-6.00652521921084));
#63669=CARTESIAN_POINT('Ctrl Pts',(-17.8679390598742,-16.541480815389,-6.01069900502764));
#63670=CARTESIAN_POINT('Ctrl Pts',(-17.7898152017669,-16.572480076405,-6.01487279084444));
#63671=CARTESIAN_POINT('Ctrl Pts',(-17.7117448631501,-16.603458101083,-6.01904371736965));
#63672=CARTESIAN_POINT('Ctrl Pts',(-17.6351421012726,-16.6383055523455,
-6.02321464389486));
#63673=CARTESIAN_POINT('Ctrl Pts',(-17.5604112612823,-16.6768539668067,
-6.02738557042007));
#63674=CARTESIAN_POINT('Ctrl Pts',(-17.4856945971113,-16.7153950689542,
-6.03155570575518));
#63675=CARTESIAN_POINT('Ctrl Pts',(-17.4128495626117,-16.7576355380395,
-6.0357258410903));
#63676=CARTESIAN_POINT('Ctrl Pts',(-17.3422580869924,-16.8033598608474,
-6.03989597642541));
#63677=CARTESIAN_POINT('Ctrl Pts',(-17.2847682206377,-16.8405978585563,
-6.04329214460284));
#63678=CARTESIAN_POINT('Ctrl Pts',(-17.2287727032861,-16.8801455850515,
-6.04668831278028));
#63679=CARTESIAN_POINT('Ctrl Pts',(-17.1744641548914,-16.9218650419685,
-6.05008448095771));
#63680=CARTESIAN_POINT('Ctrl Pts',(-17.1744641548914,-16.9218650419685,
-5.25018234058848));
#63681=CARTESIAN_POINT('Ctrl Pts',(-17.1078622797925,-16.9730281487153,
-5.25435377231504));
#63682=CARTESIAN_POINT('Ctrl Pts',(-17.0437276383886,-17.0275129995409,
-5.25852520404159));
#63683=CARTESIAN_POINT('Ctrl Pts',(-16.9824037471442,-17.0850477866369,
-5.26269663576815));
#63684=CARTESIAN_POINT('Ctrl Pts',(-16.9211031913488,-17.1425606801436,
-5.26686648014873));
#63685=CARTESIAN_POINT('Ctrl Pts',(-16.8626115968344,-17.2031208907266,
-5.27103632452931));
#63686=CARTESIAN_POINT('Ctrl Pts',(-16.8072380311628,-17.2664175144946,
-5.27520616890989));
#63687=CARTESIAN_POINT('Ctrl Pts',(-16.7518689259269,-17.329709039611,-5.27937567740234));
#63688=CARTESIAN_POINT('Ctrl Pts',(-16.6996176528133,-17.3957361932332,
-5.2835451858948));
#63689=CARTESIAN_POINT('Ctrl Pts',(-16.6507542226063,-17.4641535593445,
-5.28771469438725));
#63690=CARTESIAN_POINT('Ctrl Pts',(-16.6018800708253,-17.5325859375384,
-5.29188511774986));
#63691=CARTESIAN_POINT('Ctrl Pts',(-16.556395504268,-17.603409194585,-5.29605554111247));
#63692=CARTESIAN_POINT('Ctrl Pts',(-16.514527493463,-17.676248538027,-5.30022596447508));
#63693=CARTESIAN_POINT('Ctrl Pts',(-16.4726122042834,-17.7491701334243,
-5.30440109718101));
#63694=CARTESIAN_POINT('Ctrl Pts',(-16.4343218488226,-17.8241119583259,
-5.30857622988695));
#63695=CARTESIAN_POINT('Ctrl Pts',(-16.3998373803061,-17.9006747102711,
-5.31275136259289));
#63696=CARTESIAN_POINT('Ctrl Pts',(-16.3653298237343,-17.9772887225407,
-5.31692929063536));
#63697=CARTESIAN_POINT('Ctrl Pts',(-16.3346333926338,-18.0555253938272,
-5.32110721867783));
#63698=CARTESIAN_POINT('Ctrl Pts',(-16.307879983328,-18.134967770095,-5.32528514672029));
#63699=CARTESIAN_POINT('Ctrl Pts',(-16.2810838554183,-18.2145369962668,
-5.3294697458846));
#63700=CARTESIAN_POINT('Ctrl Pts',(-16.2582434356432,-18.2953153270739,
-5.3336543450489));
#63701=CARTESIAN_POINT('Ctrl Pts',(-16.2394399881205,-18.3768736250774,
-5.3378389442132));
#63702=CARTESIAN_POINT('Ctrl Pts',(-16.2341302779918,-18.3999040252453,
-5.33902058968222));
#63703=CARTESIAN_POINT('Ctrl Pts',(-16.2291421521855,-18.4229965796705,
-5.34020223515123));
#63704=CARTESIAN_POINT('Ctrl Pts',(-16.2244766916358,-18.4461415565825,
-5.34138388062024));
#63705=CARTESIAN_POINT('Ctrl Pts',(-16.2079546068079,-18.5281062989289,
-5.34556851501329));
#63706=CARTESIAN_POINT('Ctrl Pts',(-16.1954216323759,-18.6110338790213,
-5.34975314940633));
#63707=CARTESIAN_POINT('Ctrl Pts',(-16.1869832270606,-18.6945013429833,
-5.35393778379938));
#63708=CARTESIAN_POINT('Ctrl Pts',(-16.1785568327709,-18.7778500013414,
-5.35811646188331));
#63709=CARTESIAN_POINT('Ctrl Pts',(-16.1742134770096,-18.8617365633851,
-5.36229513996724));
#63710=CARTESIAN_POINT('Ctrl Pts',(-16.174007684269,-18.9457275683916,-5.36647381805118));
#63711=CARTESIAN_POINT('Ctrl Pts',(-16.1737982028414,-19.0312240517999,
-5.37072739593661));
#63712=CARTESIAN_POINT('Ctrl Pts',(-16.1778761703229,-19.1168282866473,
-5.37498097382205));
#63713=CARTESIAN_POINT('Ctrl Pts',(-16.1862438519478,-19.2020772082025,
-5.37923455170749));
#63714=CARTESIAN_POINT('Ctrl Pts',(-16.1944493097363,-19.2856734130638,
-5.38340566568544));
#63715=CARTESIAN_POINT('Ctrl Pts',(-16.2067795899914,-19.3689274796561,
-5.38757677966339));
#63716=CARTESIAN_POINT('Ctrl Pts',(-16.2231843067497,-19.4514041995496,
-5.39174789364134));
#63717=CARTESIAN_POINT('Ctrl Pts',(-16.2395835187467,-19.5338532435831,
-5.39591760796171));
#63718=CARTESIAN_POINT('Ctrl Pts',(-16.2600543622647,-19.6155250081436,
-5.40008732228208));
#63719=CARTESIAN_POINT('Ctrl Pts',(-16.2844950829499,-19.6959930519482,
-5.40425703660244));
#63720=CARTESIAN_POINT('Ctrl Pts',(-16.3089349339293,-19.7764582323547,
-5.40842660254649));
#63721=CARTESIAN_POINT('Ctrl Pts',(-16.3373442466931,-19.8557193372403,
-5.41259616849054));
#63722=CARTESIAN_POINT('Ctrl Pts',(-16.3695713807102,-19.9333650209191,
-5.41676573443458));
#63723=CARTESIAN_POINT('Ctrl Pts',(-16.4029315810029,-20.0137406310497,
-5.42108189717351));
#63724=CARTESIAN_POINT('Ctrl Pts',(-16.4403828646775,-20.0923846228539,
-5.42539805991243));
#63725=CARTESIAN_POINT('Ctrl Pts',(-16.4817035150007,-20.1688650474311,
-5.42971422265136));
#63726=CARTESIAN_POINT('Ctrl Pts',(-16.5216781494857,-20.2428541302221,
-5.43388978684304));
#63727=CARTESIAN_POINT('Ctrl Pts',(-16.5652736482193,-20.3148180591345,
-5.43806535103472));
#63728=CARTESIAN_POINT('Ctrl Pts',(-16.6122442629254,-20.3843940073146,
-5.44224091522641));
#63729=CARTESIAN_POINT('Ctrl Pts',(-16.6615872517182,-20.4574840712362,
-5.44662737723895));
#63730=CARTESIAN_POINT('Ctrl Pts',(-16.7146549198489,-20.5279381144878,
-5.4510138392515));
#63731=CARTESIAN_POINT('Ctrl Pts',(-16.7711149075846,-20.5953752200801,
-5.45540030126404));
#63732=CARTESIAN_POINT('Ctrl Pts',(-16.8275748953203,-20.6628123256725,
-5.45978676327659));
#63733=CARTESIAN_POINT('Ctrl Pts',(-16.8874267520076,-20.7272321203105,
-5.46417322528913));
#63734=CARTESIAN_POINT('Ctrl Pts',(-16.9502957329767,-20.788300380603,-5.46855968730168));
#63735=CARTESIAN_POINT('Ctrl Pts',(-17.0102720189371,-20.8465587997145,
-5.47274432169472));
#63736=CARTESIAN_POINT('Ctrl Pts',(-17.0732171288673,-20.9019841740837,
-5.47692895608777));
#63737=CARTESIAN_POINT('Ctrl Pts',(-17.1388325082967,-20.9542588927042,
-5.48111359048082));
#63738=CARTESIAN_POINT('Ctrl Pts',(-17.204354492355,-21.006459204733,-5.48529226856475));
#63739=CARTESIAN_POINT('Ctrl Pts',(-17.2725388396022,-21.0555174845771,
-5.48947094664869));
#63740=CARTESIAN_POINT('Ctrl Pts',(-17.3430505912408,-21.1011532616992,
-5.49364962473263));
#63741=CARTESIAN_POINT('Ctrl Pts',(-17.4148262153517,-21.1476070273285,
-5.49790320261807));
#63742=CARTESIAN_POINT('Ctrl Pts',(-17.4890131561474,-21.190514050739,-5.5021567805035));
#63743=CARTESIAN_POINT('Ctrl Pts',(-17.5652232755989,-21.2296217790709,
-5.50641035838894));
#63744=CARTESIAN_POINT('Ctrl Pts',(-17.6399559131731,-21.2679713277767,
-5.5105814723669));
#63745=CARTESIAN_POINT('Ctrl Pts',(-17.7166335547755,-21.3026673605994,
-5.51475258634485));
#63746=CARTESIAN_POINT('Ctrl Pts',(-17.7948629860233,-21.3335166740921,
-5.51892370032281));
#63747=CARTESIAN_POINT('Ctrl Pts',(-17.8730661666299,-21.3643556357998,
-5.52309341464318));
#63748=CARTESIAN_POINT('Ctrl Pts',(-17.9528196751245,-21.3913502731114,
-5.52726312896355));
#63749=CARTESIAN_POINT('Ctrl Pts',(-18.0337098641723,-21.4143553207574,
-5.53143284328393));
#63750=CARTESIAN_POINT('Ctrl Pts',(-18.1145971747999,-21.4373595497851,
-5.53560240922797));
#63751=CARTESIAN_POINT('Ctrl Pts',(-18.1966206428405,-21.4563743463907,
-5.53977197517201));
#63752=CARTESIAN_POINT('Ctrl Pts',(-18.2793523115258,-21.4713045626452,
-5.54394154111605));
#63753=CARTESIAN_POINT('Ctrl Pts',(-18.3649927236217,-21.4867597068849,
-5.54825770385497));
#63754=CARTESIAN_POINT('Ctrl Pts',(-18.4513915445807,-21.497837605271,-5.55257386659389));
#63755=CARTESIAN_POINT('Ctrl Pts',(-18.5380655626724,-21.5044908807416,
-5.55689002933282));
#63756=CARTESIAN_POINT('Ctrl Pts',(-18.6219161837412,-21.5109274264635,
-5.5610655935245));
#63757=CARTESIAN_POINT('Ctrl Pts',(-18.7060238760283,-21.5132232209822,
-5.56524115771618));
#63758=CARTESIAN_POINT('Ctrl Pts',(-18.7899505406875,-21.5113885084131,
-5.56941672190786));
#63759=CARTESIAN_POINT('Ctrl Pts',(-18.8781161416618,-21.5094611288736,
-5.5738031839204));
#63760=CARTESIAN_POINT('Ctrl Pts',(-18.9660813646935,-21.5029750554617,
-5.57818964593294));
#63761=CARTESIAN_POINT('Ctrl Pts',(-19.0533460188562,-21.492003566974,-5.58257610794549));
#63762=CARTESIAN_POINT('Ctrl Pts',(-19.140610673019,-21.4810320784863,-5.58696256995803));
#63763=CARTESIAN_POINT('Ctrl Pts',(-19.2271742005006,-21.4655753517935,
-5.59134903197057));
#63764=CARTESIAN_POINT('Ctrl Pts',(-19.3125527301388,-21.4457675790757,
-5.59573549398311));
#63765=CARTESIAN_POINT('Ctrl Pts',(-19.394002867067,-21.4268711913428,-5.59992012837616));
#63766=CARTESIAN_POINT('Ctrl Pts',(-19.4746778298126,-21.4039450190917,
-5.60410476276921));
#63767=CARTESIAN_POINT('Ctrl Pts',(-19.55414895591,-21.3770681825713,-5.60828939716226));
#63768=CARTESIAN_POINT('Ctrl Pts',(-19.6335069646959,-21.350229601901,-5.6124680752462));
#63769=CARTESIAN_POINT('Ctrl Pts',(-19.7116641083503,-21.3194516726887,
-5.61664675333015));
#63770=CARTESIAN_POINT('Ctrl Pts',(-19.7882032486926,-21.2848642288924,
-5.62082543141409));
#63771=CARTESIAN_POINT('Ctrl Pts',(-19.8661142981179,-21.2496568300237,
-5.62507900929953));
#63772=CARTESIAN_POINT('Ctrl Pts',(-19.9423482986086,-21.2105021111285,
-5.62933258718496));
#63773=CARTESIAN_POINT('Ctrl Pts',(-20.0164828014234,-21.167589732792,-5.63358616507039));
#63774=CARTESIAN_POINT('Ctrl Pts',(-20.0891800622396,-21.1255092946461,
-5.63775727904835));
#63775=CARTESIAN_POINT('Ctrl Pts',(-20.1598580881702,-21.079815837063,-5.6419283930263));
#63776=CARTESIAN_POINT('Ctrl Pts',(-20.2281415862037,-21.0307354137496,
-5.64609950700425));
#63777=CARTESIAN_POINT('Ctrl Pts',(-20.2964021710499,-20.9816714598463,
-5.65026922132462));
#63778=CARTESIAN_POINT('Ctrl Pts',(-20.3622694505382,-20.9292230656518,
-5.65443893564499));
#63779=CARTESIAN_POINT('Ctrl Pts',(-20.4253973801084,-20.8736594137782,
-5.65860864996536));
#63780=CARTESIAN_POINT('Ctrl Pts',(-20.4885230633161,-20.8180977390977,
-5.6627782159094));
#63781=CARTESIAN_POINT('Ctrl Pts',(-20.5489092456569,-20.7594213317292,
-5.66694778185344));
#63782=CARTESIAN_POINT('Ctrl Pts',(-20.6062442778983,-20.6979385338199,
-5.67111734779749));
#63783=CARTESIAN_POINT('Ctrl Pts',(-20.6655951391429,-20.6342940765832,
-5.67543351053641));
#63784=CARTESIAN_POINT('Ctrl Pts',(-20.7216759416721,-20.5676425973539,
-5.67974967327533));
#63785=CARTESIAN_POINT('Ctrl Pts',(-20.7741852955294,-20.4983647564225,
-5.68406583601425));
#63786=CARTESIAN_POINT('Ctrl Pts',(-20.8249841627079,-20.4313436338726,
-5.68824140020593));
#63787=CARTESIAN_POINT('Ctrl Pts',(-20.8724404611872,-20.3618650450197,
-5.69241696439762));
#63788=CARTESIAN_POINT('Ctrl Pts',(-20.9163256700511,-20.2903029066083,
-5.6965925285893));
#63789=CARTESIAN_POINT('Ctrl Pts',(-20.9624274164874,-20.2151263347086,
-5.70097899060184));
#63790=CARTESIAN_POINT('Ctrl Pts',(-21.0045875620259,-20.1376507144176,
-5.70536545261438));
#63791=CARTESIAN_POINT('Ctrl Pts',(-21.0425969786767,-20.0583362915701,
-5.70975191462692));
#63792=CARTESIAN_POINT('Ctrl Pts',(-21.0806063953274,-19.9790218687225,
-5.71413837663946));
#63793=CARTESIAN_POINT('Ctrl Pts',(-21.1144649298774,-19.897869208087,-5.718524838652));
#63794=CARTESIAN_POINT('Ctrl Pts',(-21.144023506431,-19.8153578044185,-5.72291130066454));
#63795=CARTESIAN_POINT('Ctrl Pts',(-21.1768030234138,-19.7238552940413,
-5.72777574688623));
#63796=CARTESIAN_POINT('Ctrl Pts',(-21.2043967060823,-19.6304025057852,
-5.73264019310792));
#63797=CARTESIAN_POINT('Ctrl Pts',(-21.2266026211961,-19.5355513454757,
-5.7375046393296));
#63798=CARTESIAN_POINT('Ctrl Pts',(-21.2488226674987,-19.4406398246877,
-5.74237218114127));
#63799=CARTESIAN_POINT('Ctrl Pts',(-21.2656479288596,-19.3443282665163,
-5.74723972295294));
#63800=CARTESIAN_POINT('Ctrl Pts',(-21.2769239065511,-19.2471914725919,
-5.75210726476461));
#63801=CARTESIAN_POINT('Ctrl Pts',(-21.2881998842426,-19.1500546786674,
-5.75697480657628));
#63802=CARTESIAN_POINT('Ctrl Pts',(-21.2939263955806,-19.0520927805187,
-5.76184234838795));
#63803=CARTESIAN_POINT('Ctrl Pts',(-21.2939992944986,-18.9539005700933,
-5.76670989019962));
#63804=CARTESIAN_POINT('Origin',(-18.734,-18.952,1.76670989022851));
#63805=CARTESIAN_POINT('',(-17.1718943060142,-16.9185142398779,-4.45010593052277));
#63806=CARTESIAN_POINT('',(-17.1769969348074,-16.9251725137323,-4.51667470085173));
#63807=CARTESIAN_POINT('',(-17.1744641548914,-16.9218650419685,1.76670989022851));
#63808=CARTESIAN_POINT('',(-21.2938494922829,-18.9508032548851,-5.03329016024732));
#63809=CARTESIAN_POINT('Ctrl Pts',(-17.1769969348074,-16.9251725137323,
-4.51667470085173));
#63810=CARTESIAN_POINT('Ctrl Pts',(-16.8552506861943,-17.1716046543912,
-4.53675462878232));
#63811=CARTESIAN_POINT('Ctrl Pts',(-16.0276178705895,-18.1629200290128,
-4.59922649227339));
#63812=CARTESIAN_POINT('Ctrl Pts',(-16.1629700483809,-20.5498410269921,
-4.70409029132494));
#63813=CARTESIAN_POINT('Ctrl Pts',(-18.6858816905041,-21.9787103574595,
-4.83126609800637));
#63814=CARTESIAN_POINT('Ctrl Pts',(-20.9008594909828,-20.8156360190963,
-4.94099937082189));
#63815=CARTESIAN_POINT('Ctrl Pts',(-21.288210216193,-19.4541225063383,-5.00834070807693));
#63816=CARTESIAN_POINT('Ctrl Pts',(-21.2903252254699,-18.9508059208324,
-5.0332901097715));
#63817=CARTESIAN_POINT('Ctrl Pts',(-21.2939997202205,-18.9508031412445,
-5.03329016239894));
#63818=CARTESIAN_POINT('Ctrl Pts',(-21.2939564765218,-18.8583078019835,
-5.03786858507833));
#63819=CARTESIAN_POINT('Ctrl Pts',(-21.2888961385929,-18.7659792628466,
-5.04244700775773));
#63820=CARTESIAN_POINT('Ctrl Pts',(-21.2788976615006,-18.6743385289801,
-5.04702543043713));
#63821=CARTESIAN_POINT('Ctrl Pts',(-21.2688681118673,-18.5824130006966,
-5.05161808160601));
#63822=CARTESIAN_POINT('Ctrl Pts',(-21.2538698091559,-18.4911798450256,
-5.05621073277489));
#63823=CARTESIAN_POINT('Ctrl Pts',(-21.2340326305246,-18.40114897993,-5.06080338394377));
#63824=CARTESIAN_POINT('Ctrl Pts',(-21.2141037578095,-18.3107019620212,
-5.06541726388461));
#63825=CARTESIAN_POINT('Ctrl Pts',(-21.1892913049386,-18.2214686542029,
-5.07003114382545));
#63826=CARTESIAN_POINT('Ctrl Pts',(-21.1597755903596,-18.1339457321084,
-5.0746450237663));
#63827=CARTESIAN_POINT('Ctrl Pts',(-21.1363775884172,-18.0645636578345,
-5.07830258630061));
#63828=CARTESIAN_POINT('Ctrl Pts',(-21.1100249393917,-17.9962560714796,
-5.08196014883493));
#63829=CARTESIAN_POINT('Ctrl Pts',(-21.0808281256644,-17.9292596866307,
-5.08561771136924));
#63830=CARTESIAN_POINT('Ctrl Pts',(-21.0474239145964,-17.8526088095457,
-5.08980234576229));
#63831=CARTESIAN_POINT('Ctrl Pts',(-21.0101982941979,-17.7774535557438,
-5.09398698015533));
#63832=CARTESIAN_POINT('Ctrl Pts',(-20.9693070771845,-17.7042010295369,
-5.09817161454838));
#63833=CARTESIAN_POINT('Ctrl Pts',(-20.9284740637572,-17.6310527692342,
-5.10235029263232));
#63834=CARTESIAN_POINT('Ctrl Pts',(-20.8839860396696,-17.5598022552459,
-5.10652897071627));
#63835=CARTESIAN_POINT('Ctrl Pts',(-20.8360465870686,-17.4908360304904,
-5.11070764880022));
#63836=CARTESIAN_POINT('Ctrl Pts',(-20.7872478542333,-17.4206336357213,
-5.11496122668565));
#63837=CARTESIAN_POINT('Ctrl Pts',(-20.7348729347517,-17.352798669429,-5.11921480457109));
#63838=CARTESIAN_POINT('Ctrl Pts',(-20.6791852047646,-17.2877120083456,
-5.12346838245653));
#63839=CARTESIAN_POINT('Ctrl Pts',(-20.6245770900889,-17.2238871791935,
-5.12763949643448));
#63840=CARTESIAN_POINT('Ctrl Pts',(-20.5667837820755,-17.1627054093254,
-5.13181061041243));
#63841=CARTESIAN_POINT('Ctrl Pts',(-20.5060958601737,-17.1044945839443,
-5.13598172439038));
#63842=CARTESIAN_POINT('Ctrl Pts',(-20.4454283026902,-17.0463032917677,
-5.14015143871076));
#63843=CARTESIAN_POINT('Ctrl Pts',(-20.3818683920876,-16.9910812823424,
-5.14432115303113));
#63844=CARTESIAN_POINT('Ctrl Pts',(-20.3157437934271,-16.9391198316952,
-5.1484908673515));
#63845=CARTESIAN_POINT('Ctrl Pts',(-20.2496215477636,-16.8871602300594,
-5.15266043329554));
#63846=CARTESIAN_POINT('Ctrl Pts',(-20.1809351577375,-16.8384612400848,
-5.15682999923958));
#63847=CARTESIAN_POINT('Ctrl Pts',(-20.1100445342429,-16.7932731901002,
-5.16099956518362));
#63848=CARTESIAN_POINT('Ctrl Pts',(-20.0366614838791,-16.7464963840235,
-5.16531572792255));
#63849=CARTESIAN_POINT('Ctrl Pts',(-19.9609167591474,-16.703482284346,-5.16963189066146));
#63850=CARTESIAN_POINT('Ctrl Pts',(-19.8832395142303,-16.6644579700185,
-5.17394805340038));
#63851=CARTESIAN_POINT('Ctrl Pts',(-19.8080925973962,-16.6267048686257,
-5.17812361759206));
#63852=CARTESIAN_POINT('Ctrl Pts',(-19.731137580502,-16.5926857570977,-5.18229918178375));
#63853=CARTESIAN_POINT('Ctrl Pts',(-19.6527837251096,-16.5625572895602,
-5.18647474597543));
#63854=CARTESIAN_POINT('Ctrl Pts',(-19.5704724027499,-16.5309071047511,
-5.19086120798797));
#63855=CARTESIAN_POINT('Ctrl Pts',(-19.4866177726054,-16.5035511069691,
-5.19524767000051));
#63856=CARTESIAN_POINT('Ctrl Pts',(-19.4017104542219,-16.4806111699446,
-5.19963413201305));
#63857=CARTESIAN_POINT('Ctrl Pts',(-19.3168031358384,-16.45767123292,-5.20402059402559));
#63858=CARTESIAN_POINT('Ctrl Pts',(-19.2308437124363,-16.439147404523,-5.20840705603813));
#63859=CARTESIAN_POINT('Ctrl Pts',(-19.1443308019265,-16.4250990060965,
-5.21279351805067));
#63860=CARTESIAN_POINT('Ctrl Pts',(-19.0590101764576,-16.4112442168689,
-5.21711952766357));
#63861=CARTESIAN_POINT('Ctrl Pts',(-18.9728228820038,-16.4016888933807,
-5.22144553727647));
#63862=CARTESIAN_POINT('Ctrl Pts',(-18.886240530398,-16.3965308022001,-5.22577154688938));
#63863=CARTESIAN_POINT('Ctrl Pts',(-18.8026253638558,-16.3915494792733,
-5.22994930375942));
#63864=CARTESIAN_POINT('Ctrl Pts',(-18.7186422840508,-16.3906689763345,
-5.23412706062947));
#63865=CARTESIAN_POINT('Ctrl Pts',(-18.6347264524453,-16.3939255752117,
-5.23830481749952));
#63866=CARTESIAN_POINT('Ctrl Pts',(-18.5508928195399,-16.3971789841283,
-5.24247848210023));
#63867=CARTESIAN_POINT('Ctrl Pts',(-18.4671267610676,-16.404561430684,-5.24665214670094));
#63868=CARTESIAN_POINT('Ctrl Pts',(-18.3838655026501,-16.4160572100764,
-5.25082581130166));
#63869=CARTESIAN_POINT('Ctrl Pts',(-18.3006608220041,-16.4275451778456,
-5.25499663980973));
#63870=CARTESIAN_POINT('Ctrl Pts',(-18.2179607144013,-16.4431408635637,
-5.2591674683178));
#63871=CARTESIAN_POINT('Ctrl Pts',(-18.1361979753704,-16.4627766794944,
-5.26333829682587));
#63872=CARTESIAN_POINT('Ctrl Pts',(-18.0544662678843,-16.4824050430121,
-5.26750754237265));
#63873=CARTESIAN_POINT('Ctrl Pts',(-17.9736716684704,-16.5060703811549,
-5.27167678791943));
#63874=CARTESIAN_POINT('Ctrl Pts',(-17.8942361136643,-16.5336541572376,
-5.27584603346621));
#63875=CARTESIAN_POINT('Ctrl Pts',(-17.8147812266298,-16.5612446463829,
-5.28001629368214));
#63876=CARTESIAN_POINT('Ctrl Pts',(-17.7366864815223,-16.5927553328241,
-5.28418655389806));
#63877=CARTESIAN_POINT('Ctrl Pts',(-17.6603570885801,-16.6280183092894,
-5.28835681411399));
#63878=CARTESIAN_POINT('Ctrl Pts',(-17.5840157549879,-16.6632868021469,
-5.29252772670794));
#63879=CARTESIAN_POINT('Ctrl Pts',(-17.5094407357015,-16.7023085494237,
-5.29669863930189));
#63880=CARTESIAN_POINT('Ctrl Pts',(-17.4370140419547,-16.7448689607018,
-5.30086955189584));
#63881=CARTESIAN_POINT('Ctrl Pts',(-17.3645257074469,-16.787465594207,-5.30504401426147));
#63882=CARTESIAN_POINT('Ctrl Pts',(-17.2941897360827,-16.8336066562081,
-5.3092184766271));
#63883=CARTESIAN_POINT('Ctrl Pts',(-17.226359753212,-16.883033860532,-5.31339293899273));
#63884=CARTESIAN_POINT('Ctrl Pts',(-17.2088933290245,-16.895761514006,-5.31446787558194));
#63885=CARTESIAN_POINT('Ctrl Pts',(-17.1915929037904,-16.9087068537485,
-5.31554281217115));
#63886=CARTESIAN_POINT('Ctrl Pts',(-17.1744641548914,-16.9218650419685,
-5.31661774876036));
#63887=CARTESIAN_POINT('',(-21.2942629789487,-18.9528355653121,-4.96670989022851));
#63888=CARTESIAN_POINT('Ctrl Pts',(-21.2939998636668,-18.952835479442,-4.96670989022851));
#63889=CARTESIAN_POINT('Ctrl Pts',(-21.2940269378476,-18.8698772454869,
-4.97085977152528));
#63890=CARTESIAN_POINT('Ctrl Pts',(-21.2900172964774,-18.7867551328103,
-4.97500965282205));
#63891=CARTESIAN_POINT('Ctrl Pts',(-21.2819493183893,-18.7038986680417,
-4.97915953411883));
#63892=CARTESIAN_POINT('Ctrl Pts',(-21.273892503302,-18.6211568449806,-4.98330367356456));
#63893=CARTESIAN_POINT('Ctrl Pts',(-21.2617885455565,-18.5386804021309,
-4.98744781301029));
#63894=CARTESIAN_POINT('Ctrl Pts',(-21.2456678375727,-18.456899329729,-4.99159195245603));
#63895=CARTESIAN_POINT('Ctrl Pts',(-21.2295645603719,-18.3752066844683,
-4.99573161098224));
#63896=CARTESIAN_POINT('Ctrl Pts',(-21.2094532518122,-18.294208373011,-4.99987126950845));
#63897=CARTESIAN_POINT('Ctrl Pts',(-21.1854159920051,-18.2143282341436,
-5.00401092803467));
#63898=CARTESIAN_POINT('Ctrl Pts',(-21.1613926712713,-18.1344944173246,
-5.00814818599592));
#63899=CARTESIAN_POINT('Ctrl Pts',(-21.1334480518403,-18.0557779336931,
-5.01228544395717));
#63900=CARTESIAN_POINT('Ctrl Pts',(-21.1017147974227,-17.9785902003445,
-5.01642270191842));
#63901=CARTESIAN_POINT('Ctrl Pts',(-21.069990038471,-17.9014231313041,-5.02055885227397));
#63902=CARTESIAN_POINT('Ctrl Pts',(-21.0344788364885,-17.8257844328049,
-5.02469500262952));
#63903=CARTESIAN_POINT('Ctrl Pts',(-20.9953624823967,-17.7520667838548,
-5.02883115298507));
#63904=CARTESIAN_POINT('Ctrl Pts',(-20.9562443890682,-17.678345857185,-5.03296748724695));
#63905=CARTESIAN_POINT('Ctrl Pts',(-20.9135210465752,-17.6065465624556,
-5.03710382150882));
#63906=CARTESIAN_POINT('Ctrl Pts',(-20.8674196102011,-17.5370368319954,
-5.0412401557707));
#63907=CARTESIAN_POINT('Ctrl Pts',(-20.8212714994527,-17.4674567279542,
-5.04538067777222));
#63908=CARTESIAN_POINT('Ctrl Pts',(-20.7717387262313,-17.4001712070023,
-5.04952119977375));
#63909=CARTESIAN_POINT('Ctrl Pts',(-20.7190913321281,-17.3355185113618,
-5.05366172177528));
#63910=CARTESIAN_POINT('Ctrl Pts',(-20.6664157771983,-17.2708312333193,
-5.05780445852121));
#63911=CARTESIAN_POINT('Ctrl Pts',(-20.6106225991452,-17.208779931402,-5.06194719526715));
#63912=CARTESIAN_POINT('Ctrl Pts',(-20.5520199344772,-17.1496672011409,
-5.06608993201309));
#63913=CARTESIAN_POINT('Ctrl Pts',(-20.493317306161,-17.0904536371683,-5.07023973538444));
#63914=CARTESIAN_POINT('Ctrl Pts',(-20.4317959684771,-17.034188968823,-5.07438953875579));
#63915=CARTESIAN_POINT('Ctrl Pts',(-20.3677981562822,-16.9811363353776,
-5.07853934212713));
#63916=CARTESIAN_POINT('Ctrl Pts',(-20.324139169833,-16.9449440949673,-5.08137031717055));
#63917=CARTESIAN_POINT('Ctrl Pts',(-20.2793283343474,-16.9102458437321,
-5.08420129221396));
#63918=CARTESIAN_POINT('Ctrl Pts',(-20.2334815623284,-16.8771132454428,
-5.08703226725737));
#63919=CARTESIAN_POINT('Ctrl Pts',(-20.1657126925719,-16.8281379601764,
-5.09121690165042));
#63920=CARTESIAN_POINT('Ctrl Pts',(-20.0954157767523,-16.7823951726099,
-5.09540153604348));
#63921=CARTESIAN_POINT('Ctrl Pts',(-20.0229321512533,-16.7401559934151,
-5.09958617043653));
#63922=CARTESIAN_POINT('Ctrl Pts',(-19.9505516972235,-16.6979769364637,
-5.10376484852047));
#63923=CARTESIAN_POINT('Ctrl Pts',(-19.8759911100092,-16.6592918118669,
-5.10794352660442));
#63924=CARTESIAN_POINT('Ctrl Pts',(-19.7996223782741,-16.6243297168797,
-5.11212220468836));
#63925=CARTESIAN_POINT('Ctrl Pts',(-19.721884791908,-16.5887409514667,-5.1163757825738));
#63926=CARTESIAN_POINT('Ctrl Pts',(-19.6422739922293,-16.5570102814914,
-5.12062936045923));
#63927=CARTESIAN_POINT('Ctrl Pts',(-19.5612105522306,-16.5293314914586,
-5.12488293834467));
#63928=CARTESIAN_POINT('Ctrl Pts',(-19.4817186851985,-16.5021893087813,
-5.12905405232262));
#63929=CARTESIAN_POINT('Ctrl Pts',(-19.4008304551545,-16.478943456341,-5.13322516630058));
#63930=CARTESIAN_POINT('Ctrl Pts',(-19.3189628776792,-16.4597282588495,
-5.13739628027853));
#63931=CARTESIAN_POINT('Ctrl Pts',(-19.2371227716601,-16.4405195092031,
-5.1415659945989));
#63932=CARTESIAN_POINT('Ctrl Pts',(-19.1543044183624,-16.4253388333996,
-5.14573570891928));
#63933=CARTESIAN_POINT('Ctrl Pts',(-19.0709381209924,-16.4142701675273,
-5.14990542323965));
#63934=CARTESIAN_POINT('Ctrl Pts',(-18.9875747901529,-16.4032018955255,
-5.1540749891837));
#63935=CARTESIAN_POINT('Ctrl Pts',(-18.9036640101516,-16.3962454022305,
-5.15824455512775));
#63936=CARTESIAN_POINT('Ctrl Pts',(-18.8196429975838,-16.3934329641448,
-5.1624141210718));
#63937=CARTESIAN_POINT('Ctrl Pts',(-18.7326679098654,-16.3905216442056,
-5.16673028381072));
#63938=CARTESIAN_POINT('Ctrl Pts',(-18.6455752209301,-16.3920512290413,
-5.17104644654963));
#63939=CARTESIAN_POINT('Ctrl Pts',(-18.5588499153532,-16.3979987376964,
-5.17536260928855));
#63940=CARTESIAN_POINT('Ctrl Pts',(-18.4749496774835,-16.4037525068827,
-5.17953817348023));
#63941=CARTESIAN_POINT('Ctrl Pts',(-18.3913937177404,-16.413640690019,-5.18371373767191));
#63942=CARTESIAN_POINT('Ctrl Pts',(-18.3086140512033,-16.4275898125371,
-5.18788930186359));
#63943=CARTESIAN_POINT('Ctrl Pts',(-18.2216533804995,-16.4422434720727,
-5.19227576387612));
#63944=CARTESIAN_POINT('Ctrl Pts',(-18.1355500550634,-16.461378961618,-5.19666222588866));
#63945=CARTESIAN_POINT('Ctrl Pts',(-18.0507884164764,-16.4848514572205,
-5.2010486879012));
#63946=CARTESIAN_POINT('Ctrl Pts',(-17.9660267778894,-16.508323952823,-5.20543514991373));
#63947=CARTESIAN_POINT('Ctrl Pts',(-17.8826073525323,-16.5361331988247,
-5.20982161192627));
#63948=CARTESIAN_POINT('Ctrl Pts',(-17.8009895271363,-16.5680764572817,
-5.21420807393881));
#63949=CARTESIAN_POINT('Ctrl Pts',(-17.723133526379,-16.5985474278393,-5.21839236074274));
#63950=CARTESIAN_POINT('Ctrl Pts',(-17.6466269368475,-16.6328931302907,
-5.22257664754668));
#63951=CARTESIAN_POINT('Ctrl Pts',(-17.571882376384,-16.6709733388491,-5.22676093435062));
#63952=CARTESIAN_POINT('Ctrl Pts',(-17.4972521228362,-16.7089953113144,
-5.23093882212142));
#63953=CARTESIAN_POINT('Ctrl Pts',(-17.4243789496429,-16.7507402336439,
-5.23511670989222));
#63954=CARTESIAN_POINT('Ctrl Pts',(-17.3536566219057,-16.7960194438374,
-5.23929459766302));
#63955=CARTESIAN_POINT('Ctrl Pts',(-17.2922215486713,-16.835352589157,-5.24292384530484));
#63956=CARTESIAN_POINT('Ctrl Pts',(-17.2324094154131,-16.8773518875695,
-5.24655309294666));
#63957=CARTESIAN_POINT('Ctrl Pts',(-17.1744641548914,-16.9218650419685,
-5.25018234058848));
#63958=CARTESIAN_POINT('Ctrl Pts',(-17.1718943060138,-16.9185142398782,
-4.45010593052279));
#63959=CARTESIAN_POINT('Ctrl Pts',(-17.1663500824386,-16.9227662676902,
-4.45045503163193));
#63960=CARTESIAN_POINT('Ctrl Pts',(-16.4898975644531,-17.4463825557267,
-4.49319606830155));
#63961=CARTESIAN_POINT('Ctrl Pts',(-15.7195029136897,-19.2278589222636,
-4.57832904053164));
#63962=CARTESIAN_POINT('Ctrl Pts',(-17.3342635996422,-21.6360321976239,
-4.70550484721307));
#63963=CARTESIAN_POINT('Ctrl Pts',(-20.2331955554845,-21.5817725214897,
-4.83268065389451));
#63964=CARTESIAN_POINT('Ctrl Pts',(-21.2762380205877,-19.8928505327429,
-4.91974900156632));
#63965=CARTESIAN_POINT('Ctrl Pts',(-21.298094862478,-18.9985742441059,-4.96442541367765));
#63966=CARTESIAN_POINT('Ctrl Pts',(-21.2979001547653,-18.9528367523378,
-4.96670989022851));
#63967=CARTESIAN_POINT('Origin',(-18.734,-18.952,1.76670989022851));
#63968=CARTESIAN_POINT('',(-17.1744641548915,-16.9218650419685,-3.65004595805791));
#63969=CARTESIAN_POINT('',(-17.1744641548914,-16.9218650419685,-3.71676815084982));
#63970=CARTESIAN_POINT('',(-17.1744641548914,-16.9218650419685,1.76670989022851));
#63971=CARTESIAN_POINT('',(-21.2939990418858,-18.954214846262,-4.23329008725046));
#63972=CARTESIAN_POINT('Ctrl Pts',(-17.1744641548914,-16.9218650419685,
-3.71676815084982));
#63973=CARTESIAN_POINT('Ctrl Pts',(-17.1078987377222,-16.9730001419821,
-3.72094076265801));
#63974=CARTESIAN_POINT('Ctrl Pts',(-17.0437863852809,-17.027462162245,-3.7251133744662));
#63975=CARTESIAN_POINT('Ctrl Pts',(-16.9824730190864,-17.0849827973123,
-3.72928598627439));
#63976=CARTESIAN_POINT('Ctrl Pts',(-16.9211916370527,-17.1424734266998,
-3.73345642143668));
#63977=CARTESIAN_POINT('Ctrl Pts',(-16.8627066771082,-17.2030191888223,
-3.73762685659898));
#63978=CARTESIAN_POINT('Ctrl Pts',(-16.8073301088088,-17.2663122678333,
-3.74179729176127));
#63979=CARTESIAN_POINT('Ctrl Pts',(-16.7519658159504,-17.3295913165336,
-3.74596680245438));
#63980=CARTESIAN_POINT('Ctrl Pts',(-16.6997088486859,-17.3956161261854,
-3.75013631314748));
#63981=CARTESIAN_POINT('Ctrl Pts',(-16.6508325531442,-17.4640438889671,
-3.75430582384059));
#63982=CARTESIAN_POINT('Ctrl Pts',(-16.601952430527,-17.5324770097288,-3.75847566101164));
#63983=CARTESIAN_POINT('Ctrl Pts',(-16.5564537715699,-17.6033130821118,
-3.76264549818268));
#63984=CARTESIAN_POINT('Ctrl Pts',(-16.5145672435831,-17.6761793857507,
-3.76681533535373));
#63985=CARTESIAN_POINT('Ctrl Pts',(-16.4726368174248,-17.7491220551721,
-3.77098954262265));
#63986=CARTESIAN_POINT('Ctrl Pts',(-16.4343263111264,-17.8240988048856,
-3.77516374989157));
#63987=CARTESIAN_POINT('Ctrl Pts',(-16.3998206964041,-17.9007117528173,
-3.7793379571605));
#63988=CARTESIAN_POINT('Ctrl Pts',(-16.365296345968,-17.9773662997259,-3.78351443092296));
#63989=CARTESIAN_POINT('Ctrl Pts',(-16.3345811690697,-18.0556583854633,
-3.78769090468543));
#63990=CARTESIAN_POINT('Ctrl Pts',(-16.3078112708355,-18.1351718354053,
-3.7918673784479));
#63991=CARTESIAN_POINT('Ctrl Pts',(-16.2809948736771,-18.2148233990543,
-3.7960511066846));
#63992=CARTESIAN_POINT('Ctrl Pts',(-16.2581375680449,-18.295700121177,-3.8002348349213));
#63993=CARTESIAN_POINT('Ctrl Pts',(-16.2393249922832,-18.3773726373784,
-3.80441856315799));
#63994=CARTESIAN_POINT('Ctrl Pts',(-16.2251740524992,-18.4388072263162,
-3.80756559029029));
#63995=CARTESIAN_POINT('Ctrl Pts',(-16.2133106237547,-18.5006918164137,
-3.81071261742259));
#63996=CARTESIAN_POINT('Ctrl Pts',(-16.2037517912764,-18.5628419315354,
-3.81385964455489));
#63997=CARTESIAN_POINT('Ctrl Pts',(-16.1910413132713,-18.645483579777,-3.818044278948));
#63998=CARTESIAN_POINT('Ctrl Pts',(-16.182360236898,-18.7289023900138,-3.82222891334111));
#63999=CARTESIAN_POINT('Ctrl Pts',(-16.1777943305987,-18.812670980335,-3.82641354773422));
#64000=CARTESIAN_POINT('Ctrl Pts',(-16.1732349233019,-18.8963203364364,
-3.83059222581822));
#64001=CARTESIAN_POINT('Ctrl Pts',(-16.1727790761929,-18.9803180282762,
-3.83477090390222));
#64002=CARTESIAN_POINT('Ctrl Pts',(-16.1764611917473,-19.0642285359493,
-3.83894958198623));
#64003=CARTESIAN_POINT('Ctrl Pts',(-16.1802093065767,-19.1496430791654,
-3.84320315987165));
#64004=CARTESIAN_POINT('Ctrl Pts',(-16.1882452624471,-19.2349668053837,
-3.84745673775707));
#64005=CARTESIAN_POINT('Ctrl Pts',(-16.2005498883094,-19.319737041342,-3.85171031564249));
#64006=CARTESIAN_POINT('Ctrl Pts',(-16.2126159649891,-19.4028638408622,
-3.8558814296205));
#64007=CARTESIAN_POINT('Ctrl Pts',(-16.2287866065493,-19.4854579433578,
-3.86005254359851));
#64008=CARTESIAN_POINT('Ctrl Pts',(-16.2489913365584,-19.5670869390747,
-3.86422365757652));
#64009=CARTESIAN_POINT('Ctrl Pts',(-16.2691892866753,-19.6486885433937,
-3.86839337189695));
#64010=CARTESIAN_POINT('Ctrl Pts',(-16.2934185263771,-19.7293252379219,
-3.87256308621738));
#64011=CARTESIAN_POINT('Ctrl Pts',(-16.3215576717043,-19.8085757483417,
-3.87673280053781));
#64012=CARTESIAN_POINT('Ctrl Pts',(-16.3496958157199,-19.8878234386882,
-3.88090236648191));
#64013=CARTESIAN_POINT('Ctrl Pts',(-16.3817434340022,-19.9656846097684,
-3.88507193242601));
#64014=CARTESIAN_POINT('Ctrl Pts',(-16.4175300086123,-20.0417553757611,
-3.88924149837011));
#64015=CARTESIAN_POINT('Ctrl Pts',(-16.4545747950371,-20.1205006960405,
-3.89355766110896));
#64016=CARTESIAN_POINT('Ctrl Pts',(-16.4956261286209,-20.1973268901834,
-3.89787382384781));
#64017=CARTESIAN_POINT('Ctrl Pts',(-16.5404425366712,-20.2718127348509,
-3.90218998658666));
#64018=CARTESIAN_POINT('Ctrl Pts',(-16.5837990549445,-20.3438722109651,
-3.90636555077841));
#64019=CARTESIAN_POINT('Ctrl Pts',(-16.6306788183654,-20.4137411050177,
-3.91054111497015));
#64020=CARTESIAN_POINT('Ctrl Pts',(-16.6808195479049,-20.4810683539772,
-3.91471667916189));
#64021=CARTESIAN_POINT('Ctrl Pts',(-16.7334927664927,-20.551796142223,-3.9191031411743));
#64022=CARTESIAN_POINT('Ctrl Pts',(-16.789764658884,-20.6197183310682,-3.9234896031867));
#64023=CARTESIAN_POINT('Ctrl Pts',(-16.8492855900872,-20.6844697957156,
-3.92787606519911));
#64024=CARTESIAN_POINT('Ctrl Pts',(-16.9088065212903,-20.7492212603631,
-3.93226252721152));
#64025=CARTESIAN_POINT('Ctrl Pts',(-16.9715760238564,-20.8108016487772,
-3.93664898922392));
#64026=CARTESIAN_POINT('Ctrl Pts',(-17.0372042845901,-20.8688944415816,
-3.94103545123633));
#64027=CARTESIAN_POINT('Ctrl Pts',(-17.0998128917647,-20.9243142988764,
-3.94522008562936));
#64028=CARTESIAN_POINT('Ctrl Pts',(-17.1652560078682,-20.9767667301136,
-3.94940472002239));
#64029=CARTESIAN_POINT('Ctrl Pts',(-17.2332206971795,-21.0259482838841,
-3.95358935441542));
#64030=CARTESIAN_POINT('Ctrl Pts',(-17.3010886471678,-21.0750598338001,
-3.95776803249934));
#64031=CARTESIAN_POINT('Ctrl Pts',(-17.3714706716863,-21.1209094865295,
-3.96194671058326));
#64032=CARTESIAN_POINT('Ctrl Pts',(-17.4440191888247,-21.1632325763699,
-3.96612538866718));
#64033=CARTESIAN_POINT('Ctrl Pts',(-17.5178680859937,-21.206314277179,-3.97037896655262));
#64034=CARTESIAN_POINT('Ctrl Pts',(-17.5939615474698,-21.2457414247196,
-3.97463254443806));
#64035=CARTESIAN_POINT('Ctrl Pts',(-17.6719001613339,-21.2812797025487,
-3.9788861223235));
#64036=CARTESIAN_POINT('Ctrl Pts',(-17.7483277830831,-21.3161290015147,
-3.98305723630144));
#64037=CARTESIAN_POINT('Ctrl Pts',(-17.8265292140563,-21.3472386721818,
-3.98722835027937));
#64038=CARTESIAN_POINT('Ctrl Pts',(-17.906102718525,-21.3744339188771,-3.9913994642573));
#64039=CARTESIAN_POINT('Ctrl Pts',(-17.9856495213358,-21.4016200399448,
-3.99556917857765));
#64040=CARTESIAN_POINT('Ctrl Pts',(-18.0665670483056,-21.4248941970682,
-3.999738892898));
#64041=CARTESIAN_POINT('Ctrl Pts',(-18.1484353715664,-21.4441304271501,
-4.00390860721835));
#64042=CARTESIAN_POINT('Ctrl Pts',(-18.2303007816012,-21.4633659727244,
-4.00807817316238));
#64043=CARTESIAN_POINT('Ctrl Pts',(-18.3131164726259,-21.4785637725468,
-4.01224773910642));
#64044=CARTESIAN_POINT('Ctrl Pts',(-18.3964505424552,-21.4896485894842,
-4.01641730505045));
#64045=CARTESIAN_POINT('Ctrl Pts',(-18.4827145353767,-21.5011231349106,
-4.02073346778939));
#64046=CARTESIAN_POINT('Ctrl Pts',(-18.5695335149128,-21.5081900216474,
-4.02504963052834));
#64047=CARTESIAN_POINT('Ctrl Pts',(-18.656422594307,-21.5108242898108,-4.02936579326728));
#64048=CARTESIAN_POINT('Ctrl Pts',(-18.7404812710781,-21.5133727469659,
-4.03354135745894));
#64049=CARTESIAN_POINT('Ctrl Pts',(-18.8246050807773,-21.5117729919952,
-4.0377169216506));
#64050=CARTESIAN_POINT('Ctrl Pts',(-18.9083568682882,-21.5060555362953,
-4.04189248584226));
#64051=CARTESIAN_POINT('Ctrl Pts',(-18.9963387594866,-21.5000493054998,
-4.04627894785484));
#64052=CARTESIAN_POINT('Ctrl Pts',(-19.0839094794603,-21.4894985417946,
-4.05066540986743));
#64053=CARTESIAN_POINT('Ctrl Pts',(-19.1705727652476,-21.474499597749,-4.05505187188001));
#64054=CARTESIAN_POINT('Ctrl Pts',(-19.2572360510348,-21.4595006537035,
-4.0594383338926));
#64055=CARTESIAN_POINT('Ctrl Pts',(-19.3429913536082,-21.4400537318181,
-4.06382479590518));
#64056=CARTESIAN_POINT('Ctrl Pts',(-19.4273615317731,-21.4163152773656,
-4.06821125791777));
#64057=CARTESIAN_POINT('Ctrl Pts',(-19.5078497129731,-21.3936690643915,
-4.07239589231081));
#64058=CARTESIAN_POINT('Ctrl Pts',(-19.5873770243866,-21.3670332665356,
-4.07658052670385));
#64059=CARTESIAN_POINT('Ctrl Pts',(-19.6655189252301,-21.336506760724,-4.08076516109689));
#64060=CARTESIAN_POINT('Ctrl Pts',(-19.7435496007498,-21.3060237056149,
-4.08494383918084));
#64061=CARTESIAN_POINT('Ctrl Pts',(-19.820198357802,-21.2716611086064,-4.08912251726478));
#64062=CARTESIAN_POINT('Ctrl Pts',(-19.8950545149195,-21.2335679725542,
-4.09330119534872));
#64063=CARTESIAN_POINT('Ctrl Pts',(-19.9712524148552,-21.1947920444153,
-4.09755477323416));
#64064=CARTESIAN_POINT('Ctrl Pts',(-20.0455923539257,-21.152150652534,-4.10180835111959));
#64065=CARTESIAN_POINT('Ctrl Pts',(-20.1176611149874,-21.1058528080795,
-4.10606192900503));
#64066=CARTESIAN_POINT('Ctrl Pts',(-20.1883326824852,-21.0604525376826,
-4.11023304298298));
#64067=CARTESIAN_POINT('Ctrl Pts',(-20.2568199436825,-21.0115365845692,
-4.11440415696092));
#64068=CARTESIAN_POINT('Ctrl Pts',(-20.3227584711504,-20.9593481313285,
-4.11857527093886));
#64069=CARTESIAN_POINT('Ctrl Pts',(-20.3886748723086,-20.9071771904272,
-4.12274498525923));
#64070=CARTESIAN_POINT('Ctrl Pts',(-20.4520438778608,-20.8517362155432,
-4.1269146995796));
#64071=CARTESIAN_POINT('Ctrl Pts',(-20.512532273786,-20.7933101181229,-4.13108441389997));
#64072=CARTESIAN_POINT('Ctrl Pts',(-20.5730185172742,-20.7348860997541,
-4.13525397984399));
#64073=CARTESIAN_POINT('Ctrl Pts',(-20.6306240246485,-20.6734774902644,
-4.13942354578802));
#64074=CARTESIAN_POINT('Ctrl Pts',(-20.6850517529254,-20.6094067266084,
-4.14359311173205));
#64075=CARTESIAN_POINT('Ctrl Pts',(-20.7413930929849,-20.5430833139418,
-4.14790927447098));
#64076=CARTESIAN_POINT('Ctrl Pts',(-20.7943286933419,-20.47390746331,-4.1522254372099));
#64077=CARTESIAN_POINT('Ctrl Pts',(-20.8435751066795,-20.4022733774286,
-4.15654159994883));
#64078=CARTESIAN_POINT('Ctrl Pts',(-20.8912173232822,-20.3329727643606,
-4.16071716414051));
#64079=CARTESIAN_POINT('Ctrl Pts',(-20.9354068051746,-20.261372036261,-4.16489272833218));
#64080=CARTESIAN_POINT('Ctrl Pts',(-20.9759325838393,-20.1878552866415,
-4.16906829252385));
#64081=CARTESIAN_POINT('Ctrl Pts',(-21.0185052232437,-20.1106253807678,
-4.17345475453641));
#64082=CARTESIAN_POINT('Ctrl Pts',(-21.0570340704736,-20.0312813353546,
-4.17784121654897));
#64083=CARTESIAN_POINT('Ctrl Pts',(-21.0913315250628,-19.9502925828359,
-4.18222767856152));
#64084=CARTESIAN_POINT('Ctrl Pts',(-21.125628979652,-19.8693038303172,-4.18661414057408));
#64085=CARTESIAN_POINT('Ctrl Pts',(-21.1556949146933,-19.7866709419479,
-4.19100060258664));
#64086=CARTESIAN_POINT('Ctrl Pts',(-21.1814026084241,-19.7028797988221,
-4.19538706459919));
#64087=CARTESIAN_POINT('Ctrl Pts',(-21.2113658472603,-19.6052182170354,
-4.20049964335886));
#64088=CARTESIAN_POINT('Ctrl Pts',(-21.235501378659,-19.5056900725396,-4.20561222211854));
#64089=CARTESIAN_POINT('Ctrl Pts',(-21.253614967081,-19.4049242957285,-4.2107248008782));
#64090=CARTESIAN_POINT('Ctrl Pts',(-21.2714816855059,-19.3055318551366,
-4.21576770033001));
#64091=CARTESIAN_POINT('Ctrl Pts',(-21.283489454374,-19.2049352741372,-4.22081059978182));
#64092=CARTESIAN_POINT('Ctrl Pts',(-21.2894978367355,-19.1037590407195,
-4.22585349923363));
#64093=CARTESIAN_POINT('Ctrl Pts',(-21.2924512874039,-19.0540253526423,
-4.22833236190591));
#64094=CARTESIAN_POINT('Ctrl Pts',(-21.2939558375883,-19.0041519285412,
-4.23081122457819));
#64095=CARTESIAN_POINT('Ctrl Pts',(-21.2939990418858,-18.954214846262,-4.23329008725046));
#64096=CARTESIAN_POINT('Ctrl Pts',(-21.2923872764654,-18.9542129983989,
-4.2332901097715));
#64097=CARTESIAN_POINT('Ctrl Pts',(-21.2874612769029,-18.3551143891762,
-4.26304769694121));
#64098=CARTESIAN_POINT('Ctrl Pts',(-20.7784813193811,-16.8950156348367,
-4.3351972196714));
#64099=CARTESIAN_POINT('Ctrl Pts',(-18.7708036927661,-16.1157767610087,
-4.42965875003148));
#64100=CARTESIAN_POINT('Ctrl Pts',(-17.5345084148665,-16.6513470387785,
-4.49436269322185));
#64101=CARTESIAN_POINT('Ctrl Pts',(-17.1769969348074,-16.9251725137323,
-4.51667470085173));
#64102=CARTESIAN_POINT('',(-21.2939989159607,-18.9496440968075,-4.16670989022851));
#64103=CARTESIAN_POINT('Ctrl Pts',(-21.2939116738757,-18.9496434105868,
-4.1667099283594));
#64104=CARTESIAN_POINT('Ctrl Pts',(-21.2957663705073,-18.7480072535544,
-4.17674049240205));
#64105=CARTESIAN_POINT('Ctrl Pts',(-21.1817725642886,-17.6962740222633,
-4.22916299200517));
#64106=CARTESIAN_POINT('Ctrl Pts',(-19.7363287120773,-16.0997001271578,
-4.32362832605963));
#64107=CARTESIAN_POINT('Ctrl Pts',(-17.839594487521,-16.4064353701673,-4.40806309607145));
#64108=CARTESIAN_POINT('Ctrl Pts',(-17.1718943060138,-16.9185142398782,
-4.45010593052279));
#64109=CARTESIAN_POINT('Ctrl Pts',(-17.1744641548914,-16.9218650419685,
-3.65004595805791));
#64110=CARTESIAN_POINT('Ctrl Pts',(-17.1077768163659,-16.9730938011375,
-3.65422167904487));
#64111=CARTESIAN_POINT('Ctrl Pts',(-17.0436659066504,-17.0275737769818,
-3.65839740003182));
#64112=CARTESIAN_POINT('Ctrl Pts',(-16.9824501210915,-17.0850042791438,
-3.66257312101877));
#64113=CARTESIAN_POINT('Ctrl Pts',(-16.9200836608067,-17.1435143039604,
-3.66682733314258));
#64114=CARTESIAN_POINT('Ctrl Pts',(-16.8607226247173,-17.2050865495661,
-3.67108154526638));
#64115=CARTESIAN_POINT('Ctrl Pts',(-16.8046620040762,-17.2693666776494,
-3.67533575739019));
#64116=CARTESIAN_POINT('Ctrl Pts',(-16.7486013834351,-17.3336468057327,
-3.67958996951399));
#64117=CARTESIAN_POINT('Ctrl Pts',(-16.6958414336857,-17.4006343840734,
-3.68384418163779));
#64118=CARTESIAN_POINT('Ctrl Pts',(-16.6466304638567,-17.4699445288448,
-3.6880983937616));
#64119=CARTESIAN_POINT('Ctrl Pts',(-16.5982243404926,-17.538121104715,-3.69228302815506));
#64120=CARTESIAN_POINT('Ctrl Pts',(-16.5530717694468,-17.6087985715455,
-3.69646766254853));
#64121=CARTESIAN_POINT('Ctrl Pts',(-16.5114409937958,-17.6816333348436,
-3.70065229694199));
#64122=CARTESIAN_POINT('Ctrl Pts',(-16.469869474401,-17.7543644268713,-3.70483097502635));
#64123=CARTESIAN_POINT('Ctrl Pts',(-16.4318100196565,-17.8292463201219,
-3.70900965311071));
#64124=CARTESIAN_POINT('Ctrl Pts',(-16.3974886040354,-17.9059051206856,
-3.71318833119507));
#64125=CARTESIAN_POINT('Ctrl Pts',(-16.3625520017101,-17.9839379751461,
-3.7174419090804));
#64126=CARTESIAN_POINT('Ctrl Pts',(-16.3314890444372,-18.0638116724915,
-3.72169548696573));
#64127=CARTESIAN_POINT('Ctrl Pts',(-16.3044899883694,-18.1451040318687,
-3.72594906485107));
#64128=CARTESIAN_POINT('Ctrl Pts',(-16.2780143616844,-18.2248203802406,
-3.73012017882945));
#64129=CARTESIAN_POINT('Ctrl Pts',(-16.2554466207296,-18.3059004177645,
-3.73429129280783));
#64130=CARTESIAN_POINT('Ctrl Pts',(-16.2369175937362,-18.3879260187458,
-3.73846240678621));
#64131=CARTESIAN_POINT('Ctrl Pts',(-16.2183947843368,-18.4699240952445,
-3.74263212110702));
#64132=CARTESIAN_POINT('Ctrl Pts',(-16.2039080986716,-18.5528666566986,
-3.74680183542783));
#64133=CARTESIAN_POINT('Ctrl Pts',(-16.1935378668542,-18.6363227121694,
-3.75097154974863));
#64134=CARTESIAN_POINT('Ctrl Pts',(-16.1831680040541,-18.7197757979158,
-3.75514111569312));
#64135=CARTESIAN_POINT('Ctrl Pts',(-16.1769143597415,-18.8037418847219,
-3.75931068163761));
#64136=CARTESIAN_POINT('Ctrl Pts',(-16.174805548368,-18.8877835010606,-3.76348024758209));
#64137=CARTESIAN_POINT('Ctrl Pts',(-16.1726225937887,-18.9747799169337,
-3.7677964103205));
#64138=CARTESIAN_POINT('Ctrl Pts',(-16.1748813730051,-19.0618567451386,
-3.77211257305891));
#64139=CARTESIAN_POINT('Ctrl Pts',(-16.1815548449752,-19.1485292105273,
-3.77642873579733));
#64140=CARTESIAN_POINT('Ctrl Pts',(-16.1880109292993,-19.2323783294909,
-3.78060429998945));
#64141=CARTESIAN_POINT('Ctrl Pts',(-16.1985983999138,-19.3158485639561,
-3.78477986418157));
#64142=CARTESIAN_POINT('Ctrl Pts',(-16.2132401674605,-19.3985085292081,
-3.78895542837369));
#64143=CARTESIAN_POINT('Ctrl Pts',(-16.2286214558734,-19.485343452771,-3.79334189038525));
#64144=CARTESIAN_POINT('Ctrl Pts',(-16.2484772384201,-19.5712835336828,
-3.7977283523968));
#64145=CARTESIAN_POINT('Ctrl Pts',(-16.272658640717,-19.6558456599874,-3.80211481440836));
#64146=CARTESIAN_POINT('Ctrl Pts',(-16.2968400430139,-19.7404077862919,
-3.80650127641991));
#64147=CARTESIAN_POINT('Ctrl Pts',(-16.3253468050044,-19.8235914337677,
-3.81088773843147));
#64148=CARTESIAN_POINT('Ctrl Pts',(-16.3579723492966,-19.9049389293615,
-3.81527420044303));
#64149=CARTESIAN_POINT('Ctrl Pts',(-16.3890967439393,-19.9825435061125,
-3.81945883483596));
#64150=CARTESIAN_POINT('Ctrl Pts',(-16.4240850782656,-20.0587660450939,
-3.8236434692289));
#64151=CARTESIAN_POINT('Ctrl Pts',(-16.4627936385718,-20.133195015147,-3.82782810362183));
#64152=CARTESIAN_POINT('Ctrl Pts',(-16.5014471020335,-20.2075180447734,
-3.83200678170565));
#64153=CARTESIAN_POINT('Ctrl Pts',(-16.5438100629347,-20.280052171735,-3.83618545978947));
#64154=CARTESIAN_POINT('Ctrl Pts',(-16.5896904513639,-20.3504050055789,
-3.84036413787329));
#64155=CARTESIAN_POINT('Ctrl Pts',(-16.6363932127838,-20.4220188634104,
-3.84461771575875));
#64156=CARTESIAN_POINT('Ctrl Pts',(-16.6867405623481,-20.49137201211,-3.84887129364422));
#64157=CARTESIAN_POINT('Ctrl Pts',(-16.7404804948179,-20.5580759578732,
-3.85312487152969));
#64158=CARTESIAN_POINT('Ctrl Pts',(-16.79317857383,-20.6234867174835,-3.85729598550753));
#64159=CARTESIAN_POINT('Ctrl Pts',(-16.8491385640368,-20.6863497027056,
-3.86146709948537));
#64160=CARTESIAN_POINT('Ctrl Pts',(-16.9080797027391,-20.7463285841926,
-3.86563821346321));
#64161=CARTESIAN_POINT('Ctrl Pts',(-16.967001063173,-20.8062873391867,-3.86980792778346));
#64162=CARTESIAN_POINT('Ctrl Pts',(-17.028901263212,-20.8633635846445,-3.87397764210372));
#64163=CARTESIAN_POINT('Ctrl Pts',(-17.0934613888496,-20.9172564884321,
-3.87814735642397));
#64164=CARTESIAN_POINT('Ctrl Pts',(-17.1580192171609,-20.9711474744791,
-3.88231692236791));
#64165=CARTESIAN_POINT('Ctrl Pts',(-17.2252364291759,-21.0218550499285,
-3.88648648831184));
#64166=CARTESIAN_POINT('Ctrl Pts',(-17.2947606690316,-21.0691183595145,
-3.89065605425577));
#64167=CARTESIAN_POINT('Ctrl Pts',(-17.3667292953974,-21.1180433887629,
-3.89497221699483));
#64168=CARTESIAN_POINT('Ctrl Pts',(-17.4411697620694,-21.1632771484776,
-3.89928837973389));
#64169=CARTESIAN_POINT('Ctrl Pts',(-17.5176598130617,-21.2045799763025,
-3.90360454247294));
#64170=CARTESIAN_POINT('Ctrl Pts',(-17.5916582086839,-21.2445373688529,
-3.90778010666451));
#64171=CARTESIAN_POINT('Ctrl Pts',(-17.6675742634434,-21.2808158363469,
-3.91195567085607));
#64172=CARTESIAN_POINT('Ctrl Pts',(-17.7450035240558,-21.3132466983714,
-3.91613123504764));
#64173=CARTESIAN_POINT('Ctrl Pts',(-17.8263435525583,-21.3473155661427,
-3.92051769706044));
#64174=CARTESIAN_POINT('Ctrl Pts',(-17.9093531188135,-21.3771377310941,
-3.92490415907325));
#64175=CARTESIAN_POINT('Ctrl Pts',(-17.9935454192395,-21.4025768736832,
-3.92929062108605));
#64176=CARTESIAN_POINT('Ctrl Pts',(-18.0777377196656,-21.4280160162723,
-3.93367708309886));
#64177=CARTESIAN_POINT('Ctrl Pts',(-18.1631121727114,-21.4490720714144,
-3.93806354511166));
#64178=CARTESIAN_POINT('Ctrl Pts',(-18.249172131343,-21.4656710082613,-3.94245000712447));
#64179=CARTESIAN_POINT('Ctrl Pts',(-18.3312723437006,-21.4815062034173,
-3.94663464151747));
#64180=CARTESIAN_POINT('Ctrl Pts',(-18.4143019582715,-21.4933443659487,
-3.95081927591047));
#64181=CARTESIAN_POINT('Ctrl Pts',(-18.4978371529754,-21.5010835823262,
-3.95500391030347));
#64182=CARTESIAN_POINT('Ctrl Pts',(-18.5812534456692,-21.5088117828872,
-3.95918258838737));
#64183=CARTESIAN_POINT('Ctrl Pts',(-18.6651734349296,-21.5124525840588,
-3.96336126647127));
#64184=CARTESIAN_POINT('Ctrl Pts',(-18.7491632186829,-21.511955092731,-3.96753994455516));
#64185=CARTESIAN_POINT('Ctrl Pts',(-18.8346584589487,-21.5114486842287,
-3.97179352244061));
#64186=CARTESIAN_POINT('Ctrl Pts',(-18.920225547037,-21.5066540748902,-3.97604710032606));
#64187=CARTESIAN_POINT('Ctrl Pts',(-19.0054014154825,-21.4975728769128,
-3.9803006782115));
#64188=CARTESIAN_POINT('Ctrl Pts',(-19.0889259835099,-21.4886677356789,
-3.9844717921894));
#64189=CARTESIAN_POINT('Ctrl Pts',(-19.1720738871333,-21.4756407813847,
-3.9886429061673));
#64190=CARTESIAN_POINT('Ctrl Pts',(-19.2544103550736,-21.4585460423324,
-3.9928140201452));
#64191=CARTESIAN_POINT('Ctrl Pts',(-19.3367191942171,-21.4414570395848,
-3.99698373446553));
#64192=CARTESIAN_POINT('Ctrl Pts',(-19.4182166883875,-21.4203030563999,
-4.00115344878585));
#64193=CARTESIAN_POINT('Ctrl Pts',(-19.4984772632651,-21.3951894142597,
-4.00532316310618));
#64194=CARTESIAN_POINT('Ctrl Pts',(-19.5787349821266,-21.3700766657708,
-4.00949272905015));
#64195=CARTESIAN_POINT('Ctrl Pts',(-19.6577554304208,-21.3410046766653,
-4.01366229499412));
#64196=CARTESIAN_POINT('Ctrl Pts',(-19.7351285466046,-21.3081285264546,
-4.0178318609381));
#64197=CARTESIAN_POINT('Ctrl Pts',(-19.815222006106,-21.2740964913586,-4.02214802367708));
#64198=CARTESIAN_POINT('Ctrl Pts',(-19.8935496523612,-21.2359880155544,
-4.02646418641606));
#64199=CARTESIAN_POINT('Ctrl Pts',(-19.9696814080998,-21.1940284248146,
-4.03078034915504));
#64200=CARTESIAN_POINT('Ctrl Pts',(-20.0433331799007,-21.1534356633309,
-4.03495591334667));
#64201=CARTESIAN_POINT('Ctrl Pts',(-20.1149295504515,-21.1092391216322,
-4.03913147753829));
#64202=CARTESIAN_POINT('Ctrl Pts',(-20.1841097633271,-21.061687577416,-4.04330704172992));
#64203=CARTESIAN_POINT('Ctrl Pts',(-20.2567841042977,-21.0117343177424,
-4.04769350374258));
#64204=CARTESIAN_POINT('Ctrl Pts',(-20.3267913293724,-20.9580785813378,
-4.05207996575524));
#64205=CARTESIAN_POINT('Ctrl Pts',(-20.3937533178434,-20.9010559057933,
-4.0564664277679));
#64206=CARTESIAN_POINT('Ctrl Pts',(-20.4607153063143,-20.8440332302489,
-4.06085288978057));
#64207=CARTESIAN_POINT('Ctrl Pts',(-20.524631688673,-20.7836440693278,-4.06523935179323));
#64208=CARTESIAN_POINT('Ctrl Pts',(-20.5851713910718,-20.7202659530956,
-4.06962581380589));
#64209=CARTESIAN_POINT('Ctrl Pts',(-20.6421808499863,-20.66058359639,-4.07375648865202));
#64210=CARTESIAN_POINT('Ctrl Pts',(-20.6964202744403,-20.5980163329693,
-4.07788716349815));
#64211=CARTESIAN_POINT('Ctrl Pts',(-20.747578131795,-20.5328551822216,-4.08201783834428));
#64212=CARTESIAN_POINT('Ctrl Pts',(-20.7986699217385,-20.467778183328,-4.08614317866296));
#64213=CARTESIAN_POINT('Ctrl Pts',(-20.8466877493678,-20.4001143092104,
-4.09026851898165));
#64214=CARTESIAN_POINT('Ctrl Pts',(-20.8913569516645,-20.3301911997632,
-4.09439385930034));
#64215=CARTESIAN_POINT('Ctrl Pts',(-20.9359826817961,-20.2603361396387,
-4.09851518482882));
#64216=CARTESIAN_POINT('Ctrl Pts',(-20.9772659998208,-20.188226602647,-4.10263651035731));
#64217=CARTESIAN_POINT('Ctrl Pts',(-21.0149735460513,-20.1142218730579,
-4.10675783588579));
#64218=CARTESIAN_POINT('Ctrl Pts',(-21.0526563884391,-20.0402656271644,
-4.11087646135587));
#64219=CARTESIAN_POINT('Ctrl Pts',(-21.0867678956212,-19.9644170734847,
-4.11499508682595));
#64220=CARTESIAN_POINT('Ctrl Pts',(-21.1171197545789,-19.8870616211436,
-4.11911371229603));
#64221=CARTESIAN_POINT('Ctrl Pts',(-21.1474714047475,-19.8097067009274,
-4.12323230943426));
#64222=CARTESIAN_POINT('Ctrl Pts',(-21.1740632676919,-19.730845335542,-4.12735090657249));
#64223=CARTESIAN_POINT('Ctrl Pts',(-21.1967549321189,-19.6508834983916,
-4.13146950371072));
#64224=CARTESIAN_POINT('Ctrl Pts',(-21.2194452848828,-19.5709262833344,
-4.13558786277862));
#64225=CARTESIAN_POINT('Ctrl Pts',(-21.238235765403,-19.4898691801177,-4.13970622184653));
#64226=CARTESIAN_POINT('Ctrl Pts',(-21.2530362470693,-19.4081319830388,
-4.14382458091443));
#64227=CARTESIAN_POINT('Ctrl Pts',(-21.2678499327185,-19.3263218655936,
-4.14794661410211));
#64228=CARTESIAN_POINT('Ctrl Pts',(-21.2786664327327,-19.2438309098082,
-4.15206864728979));
#64229=CARTESIAN_POINT('Ctrl Pts',(-21.2854471635996,-19.1610869947161,
-4.15619068047747));
#64230=CARTESIAN_POINT('Ctrl Pts',(-21.2912151852698,-19.090700969273,-4.15969708372782));
#64231=CARTESIAN_POINT('Ctrl Pts',(-21.2940637843831,-19.0201321760509,
-4.16320348697816));
#64232=CARTESIAN_POINT('Ctrl Pts',(-21.2939989159607,-18.9496440968075,
-4.16670989022851));
#64233=CARTESIAN_POINT('Origin',(-18.734,-18.952,1.76670989022851));
#64234=CARTESIAN_POINT('',(-17.1767158332877,-16.9247660182631,-2.85017128494026));
#64235=CARTESIAN_POINT('',(-17.1744641548914,-16.9218650419685,-2.9166563088035));
#64236=CARTESIAN_POINT('',(-17.1744641548914,-16.9218650419685,1.76670989022851));
#64237=CARTESIAN_POINT('',(-21.2939999971965,-18.9521198080496,-3.43329010980363));
#64238=CARTESIAN_POINT('Ctrl Pts',(-17.1744641548914,-16.9218650419685,
-2.9166563088035));
#64239=CARTESIAN_POINT('Ctrl Pts',(-17.1375640854123,-16.9502114239723,
-2.91898053846395));
#64240=CARTESIAN_POINT('Ctrl Pts',(-17.1014709448253,-16.9795381858104,
-2.9213047681244));
#64241=CARTESIAN_POINT('Ctrl Pts',(-17.0662376770538,-17.0097927931961,
-2.92362899778485));
#64242=CARTESIAN_POINT('Ctrl Pts',(-17.0028023176014,-17.0642643769008,
-2.92781363217407));
#64243=CARTESIAN_POINT('Ctrl Pts',(-16.9419203976444,-17.1219484370566,
-2.93199826656328));
#64244=CARTESIAN_POINT('Ctrl Pts',(-16.8839351856056,-17.1825763134456,
-2.9361829009525));
#64245=CARTESIAN_POINT('Ctrl Pts',(-16.8260325083402,-17.2431178935555,
-2.94036157903253));
#64246=CARTESIAN_POINT('Ctrl Pts',(-16.7710186644549,-17.3065946373125,
-2.94454025711256));
#64247=CARTESIAN_POINT('Ctrl Pts',(-16.7192032202856,-17.3726982756761,
-2.9487189351926));
#64248=CARTESIAN_POINT('Ctrl Pts',(-16.6664590214574,-17.4399867743277,
-2.952972513079));
#64249=CARTESIAN_POINT('Ctrl Pts',(-16.6170293785859,-17.5099969539576,
-2.95722609096541));
#64250=CARTESIAN_POINT('Ctrl Pts',(-16.5712008555433,-17.5823650629685,
-2.96147966885181));
#64251=CARTESIAN_POINT('Ctrl Pts',(-16.5262608079009,-17.6533301748861,
-2.96565078282569));
#64252=CARTESIAN_POINT('Ctrl Pts',(-16.4847837540971,-17.7265621993711,
-2.96982189679958));
#64253=CARTESIAN_POINT('Ctrl Pts',(-16.4469976092765,-17.8016869709401,
-2.97399301077346));
#64254=CARTESIAN_POINT('Ctrl Pts',(-16.4092241439622,-17.8767865336655,
-2.97816272508971));
#64255=CARTESIAN_POINT('Ctrl Pts',(-16.3751393344499,-17.9537771714644,
-2.98233243940597));
#64256=CARTESIAN_POINT('Ctrl Pts',(-16.3449251982367,-18.0322600413271,
-2.98650215372222));
#64257=CARTESIAN_POINT('Ctrl Pts',(-16.3147121371724,-18.1107401184316,
-2.9906717196621));
#64258=CARTESIAN_POINT('Ctrl Pts',(-16.2883696400365,-18.1907118923997,
-2.99484128560198));
#64259=CARTESIAN_POINT('Ctrl Pts',(-16.2660311035624,-18.2717577444641,
-2.99901085154186));
#64260=CARTESIAN_POINT('Ctrl Pts',(-16.2429071716547,-18.355653068883,-3.00332701428556));
#64261=CARTESIAN_POINT('Ctrl Pts',(-16.2240741377505,-18.4406988974033,
-3.00764317702926));
#64262=CARTESIAN_POINT('Ctrl Pts',(-16.2096228114113,-18.5264182690326,
-3.01195933977297));
#64263=CARTESIAN_POINT('Ctrl Pts',(-16.1956422355373,-18.6093453409713,
-3.01613490396041));
#64264=CARTESIAN_POINT('Ctrl Pts',(-16.185762291265,-18.6929022752325,-3.02031046814786));
#64265=CARTESIAN_POINT('Ctrl Pts',(-16.1800123293529,-18.7766518372414,
-3.0244860323353));
#64266=CARTESIAN_POINT('Ctrl Pts',(-16.173971950515,-18.8646313908073,-3.02887249435713));
#64267=CARTESIAN_POINT('Ctrl Pts',(-16.172489739197,-18.9528229589758,-3.03325895637896));
#64268=CARTESIAN_POINT('Ctrl Pts',(-16.1755378747839,-19.0407217776812,
-3.0376454184008));
#64269=CARTESIAN_POINT('Ctrl Pts',(-16.1785860103708,-19.1286205963865,
-3.04203188042263));
#64270=CARTESIAN_POINT('Ctrl Pts',(-16.1861643670755,-19.216226094126,-3.04641834244446));
#64271=CARTESIAN_POINT('Ctrl Pts',(-16.1981829862586,-19.3030442604849,
-3.05080480446629));
#64272=CARTESIAN_POINT('Ctrl Pts',(-16.2096486109408,-19.3858677941965,
-3.05498943886226));
#64273=CARTESIAN_POINT('Ctrl Pts',(-16.2251975483163,-19.4682831419491,
-3.05917407325822));
#64274=CARTESIAN_POINT('Ctrl Pts',(-16.2447897023432,-19.5498562486412,
-3.06335870765419));
#64275=CARTESIAN_POINT('Ctrl Pts',(-16.264353969364,-19.6313132461135,-3.06753738574109));
#64276=CARTESIAN_POINT('Ctrl Pts',(-16.2879499152426,-19.7119299402847,
-3.07171606382799));
#64277=CARTESIAN_POINT('Ctrl Pts',(-16.3154858968853,-19.7912791746703,
-3.07589474191489));
#64278=CARTESIAN_POINT('Ctrl Pts',(-16.3435154411845,-19.872050686984,-3.0801483197996));
#64279=CARTESIAN_POINT('Ctrl Pts',(-16.3756275947397,-19.9515083765662,
-3.0844018976843));
#64280=CARTESIAN_POINT('Ctrl Pts',(-16.411671611611,-20.0292143967114,-3.088655475569));
#64281=CARTESIAN_POINT('Ctrl Pts',(-16.4470168449129,-20.105413934094,-3.09282658954999));
#64282=CARTESIAN_POINT('Ctrl Pts',(-16.4861426458315,-20.1799286784567,
-3.09699770353098));
#64283=CARTESIAN_POINT('Ctrl Pts',(-16.528857766552,-20.252364460551,-3.10116881751197));
#64284=CARTESIAN_POINT('Ctrl Pts',(-16.5715585538015,-20.3247759361195,
-3.1053385318354));
#64285=CARTESIAN_POINT('Ctrl Pts',(-16.6178460353525,-20.3951094389607,
-3.10950824615883));
#64286=CARTESIAN_POINT('Ctrl Pts',(-16.6674833699697,-20.4629960350075,
-3.11367796048227));
#64287=CARTESIAN_POINT('Ctrl Pts',(-16.7171189382778,-20.5308802153581,
-3.11784752642939));
#64288=CARTESIAN_POINT('Ctrl Pts',(-16.7701038504332,-20.596317291184,-3.12201709237651));
#64289=CARTESIAN_POINT('Ctrl Pts',(-16.8261591602626,-20.6589690478243,
-3.12618665832363));
#64290=CARTESIAN_POINT('Ctrl Pts',(-16.8841853055431,-20.7238235628371,
-3.13050282105897));
#64291=CARTESIAN_POINT('Ctrl Pts',(-16.9455014243904,-20.7856928577369,
-3.13481898379432));
#64292=CARTESIAN_POINT('Ctrl Pts',(-17.0097556215867,-20.8442424061177,
-3.13913514652966));
#64293=CARTESIAN_POINT('Ctrl Pts',(-17.0719167451653,-20.9008847092073,
-3.14331071072443));
#64294=CARTESIAN_POINT('Ctrl Pts',(-17.1368270773973,-20.9544199625766,
-3.14748627491921));
#64295=CARTESIAN_POINT('Ctrl Pts',(-17.2041348602072,-21.0045868200996,
-3.15166183911398));
#64296=CARTESIAN_POINT('Ctrl Pts',(-17.2748421989537,-21.0572874862135,
-3.15604830111961));
#64297=CARTESIAN_POINT('Ctrl Pts',(-17.3481950580325,-21.1062702142998,
-3.16043476312523));
#64298=CARTESIAN_POINT('Ctrl Pts',(-17.4237539519795,-21.1512851778809,
-3.16482122513085));
#64299=CARTESIAN_POINT('Ctrl Pts',(-17.4993128459265,-21.1963001414621,
-3.16920768713647));
#64300=CARTESIAN_POINT('Ctrl Pts',(-17.5770772261123,-21.2373471369617,
-3.1735941491421));
#64301=CARTESIAN_POINT('Ctrl Pts',(-17.6565830150582,-21.2742344068933,
-3.17798061114772));
#64302=CARTESIAN_POINT('Ctrl Pts',(-17.7324306249074,-21.3094244389056,
-3.18216524554016));
#64303=CARTESIAN_POINT('Ctrl Pts',(-17.8101452346756,-21.3409601078314,
-3.1863498799326));
#64304=CARTESIAN_POINT('Ctrl Pts',(-17.889340169487,-21.3686401823022,-3.19053451432504));
#64305=CARTESIAN_POINT('Ctrl Pts',(-17.968422380111,-21.3962808576131,-3.19471319240837));
#64306=CARTESIAN_POINT('Ctrl Pts',(-18.0489802999383,-21.4200766888,-3.19889187049171));
#64307=CARTESIAN_POINT('Ctrl Pts',(-18.1306051532971,-21.4398735214983,
-3.20307054857504));
#64308=CARTESIAN_POINT('Ctrl Pts',(-18.2136930735046,-21.4600251981986,
-3.20732412646063));
#64309=CARTESIAN_POINT('Ctrl Pts',(-18.2978861156725,-21.4760328992744,
-3.21157770434622));
#64310=CARTESIAN_POINT('Ctrl Pts',(-18.3827345240933,-21.4877863800873,
-3.21583128223181));
#64311=CARTESIAN_POINT('Ctrl Pts',(-18.4659379805337,-21.4993119967374,
-3.22000239620915));
#64312=CARTESIAN_POINT('Ctrl Pts',(-18.5497711422163,-21.5067468078098,
-3.22417351018649));
#64313=CARTESIAN_POINT('Ctrl Pts',(-18.6337990563677,-21.5100382661124,
-3.22834462416383));
#64314=CARTESIAN_POINT('Ctrl Pts',(-18.717798774141,-21.5133286199344,-3.23251433848359));
#64315=CARTESIAN_POINT('Ctrl Pts',(-18.801992655297,-21.5124783642369,-3.23668405280335));
#64316=CARTESIAN_POINT('Ctrl Pts',(-18.8859422870023,-21.5074869480043,
-3.24085376712312));
#64317=CARTESIAN_POINT('Ctrl Pts',(-18.9698889314194,-21.5024957093878,
-3.24502333306655));
#64318=CARTESIAN_POINT('Ctrl Pts',(-19.0535908844953,-21.4933636313811,
-3.24919289900999));
#64319=CARTESIAN_POINT('Ctrl Pts',(-19.1366127729516,-21.4801421943902,
-3.25336246495342));
#64320=CARTESIAN_POINT('Ctrl Pts',(-19.2225536086144,-21.4664559079809,
-3.25767862769307));
#64321=CARTESIAN_POINT('Ctrl Pts',(-19.3077651468763,-21.4483874314135,
-3.26199479043271));
#64322=CARTESIAN_POINT('Ctrl Pts',(-19.3917756297605,-21.4260515800794,
-3.26631095317236));
#64323=CARTESIAN_POINT('Ctrl Pts',(-19.4730494799758,-21.4044433167598,
-3.27048651736344));
#64324=CARTESIAN_POINT('Ctrl Pts',(-19.5531988875815,-21.378841616957,-3.27466208155452));
#64325=CARTESIAN_POINT('Ctrl Pts',(-19.6318137018703,-21.3494007918439,
-3.2788376457456));
#64326=CARTESIAN_POINT('Ctrl Pts',(-19.7143991635779,-21.3184729806291,
-3.28322410775952));
#64327=CARTESIAN_POINT('Ctrl Pts',(-19.7952903977543,-21.2833082561225,
-3.28761056977345));
#64328=CARTESIAN_POINT('Ctrl Pts',(-19.8740394547188,-21.2441409297171,
-3.29199703178738));
#64329=CARTESIAN_POINT('Ctrl Pts',(-19.9527885116833,-21.2049736033117,
-3.2963834938013));
#64330=CARTESIAN_POINT('Ctrl Pts',(-20.0293949232976,-21.161804026126,-3.30076995581523));
#64331=CARTESIAN_POINT('Ctrl Pts',(-20.103446255522,-21.1149186191895,-3.30515641782916));
#64332=CARTESIAN_POINT('Ctrl Pts',(-20.1740903761505,-21.070190479346,-3.30934105222176));
#64333=CARTESIAN_POINT('Ctrl Pts',(-20.2426723273843,-21.0219144506012,
-3.31352568661436));
#64334=CARTESIAN_POINT('Ctrl Pts',(-20.3088136057118,-20.97030674261,-3.31771032100697));
#64335=CARTESIAN_POINT('Ctrl Pts',(-20.374860740116,-20.9187724918035,-3.32188899909045));
#64336=CARTESIAN_POINT('Ctrl Pts',(-20.4384737424745,-20.8639162618918,
-3.32606767717394));
#64337=CARTESIAN_POINT('Ctrl Pts',(-20.4993017308436,-20.8059983276909,
-3.33024635525743));
#64338=CARTESIAN_POINT('Ctrl Pts',(-20.5612200171964,-20.7470422561363,
-3.33449993314298));
#64339=CARTESIAN_POINT('Ctrl Pts',(-20.6202520574043,-20.6849138964936,
-3.33875351102852));
#64340=CARTESIAN_POINT('Ctrl Pts',(-20.6760617089388,-20.6199317488056,
-3.34300708891407));
#64341=CARTESIAN_POINT('Ctrl Pts',(-20.7307893814671,-20.5562094068616,
-3.34717820289155));
#64342=CARTESIAN_POINT('Ctrl Pts',(-20.7824181813927,-20.4897433069906,
-3.35134931686903));
#64343=CARTESIAN_POINT('Ctrl Pts',(-20.8306684931562,-20.4208707328441,
-3.3555204308465));
#64344=CARTESIAN_POINT('Ctrl Pts',(-20.8789026140616,-20.352021269555,-3.3596901451664));
#64345=CARTESIAN_POINT('Ctrl Pts',(-20.923760234583,-20.2807673121879,-3.36385985948629));
#64346=CARTESIAN_POINT('Ctrl Pts',(-20.965003586852,-20.2074771983009,-3.36802957380619));
#64347=CARTESIAN_POINT('Ctrl Pts',(-21.0062454715054,-20.1341896923909,
-3.37219913974974));
#64348=CARTESIAN_POINT('Ctrl Pts',(-21.0438731187515,-20.0588665753507,
-3.3763687056933));
#64349=CARTESIAN_POINT('Ctrl Pts',(-21.0776941561667,-19.9819017925755,
-3.38053827163685));
#64350=CARTESIAN_POINT('Ctrl Pts',(-21.1127042995432,-19.9022310229647,
-3.38485443437633));
#64351=CARTESIAN_POINT('Ctrl Pts',(-21.1436349596428,-19.8208014806364,
-3.38917059711581));
#64352=CARTESIAN_POINT('Ctrl Pts',(-21.1703273243944,-19.7380719867856,
-3.39348675985529));
#64353=CARTESIAN_POINT('Ctrl Pts',(-21.1961501881654,-19.6580373975152,
-3.39766232404647));
#64354=CARTESIAN_POINT('Ctrl Pts',(-21.2180065643708,-19.5767867151054,
-3.40183788823765));
#64355=CARTESIAN_POINT('Ctrl Pts',(-21.2358041974883,-19.4947483371046,
-3.40601345242883));
#64356=CARTESIAN_POINT('Ctrl Pts',(-21.2545007467516,-19.4085663956271,
-3.41039991444246));
#64357=CARTESIAN_POINT('Ctrl Pts',(-21.2687176692139,-19.3215156705805,
-3.41478637645609));
#64358=CARTESIAN_POINT('Ctrl Pts',(-21.2784095170101,-19.2340996450695,
-3.41917283846971));
#64359=CARTESIAN_POINT('Ctrl Pts',(-21.2881013648063,-19.1466836195585,
-3.42355930048334));
#64360=CARTESIAN_POINT('Ctrl Pts',(-21.293268179777,-19.0589028772671,-3.42794576249697));
#64361=CARTESIAN_POINT('Ctrl Pts',(-21.2939275539577,-18.9712592442245,
-3.43233222451059));
#64362=CARTESIAN_POINT('Ctrl Pts',(-21.2939755504833,-18.9648795739236,
-3.43265151959756));
#64363=CARTESIAN_POINT('Ctrl Pts',(-21.2939996986147,-18.958499723977,-3.43297081468453));
#64364=CARTESIAN_POINT('Ctrl Pts',(-21.2939999971965,-18.9521198086916,
-3.4332901097715));
#64365=CARTESIAN_POINT('Ctrl Pts',(-21.2939999971965,-18.9521198080496,
-3.43329010980363));
#64366=CARTESIAN_POINT('Ctrl Pts',(-21.294003905102,-18.8686175883755,-3.43746913841141));
#64367=CARTESIAN_POINT('Ctrl Pts',(-21.2899179933662,-18.784957797327,-3.44164816701919));
#64368=CARTESIAN_POINT('Ctrl Pts',(-21.2817219740999,-18.7015748760837,
-3.44582719562697));
#64369=CARTESIAN_POINT('Ctrl Pts',(-21.2735376207105,-18.6183106386626,
-3.45000027597723));
#64370=CARTESIAN_POINT('Ctrl Pts',(-21.2612548239782,-18.5353229435677,
-3.45417335632749));
#64371=CARTESIAN_POINT('Ctrl Pts',(-21.2449053023278,-18.4530465324881,
-3.45834643667775));
#64372=CARTESIAN_POINT('Ctrl Pts',(-21.228391285294,-18.3699423241145,-3.46256150311585));
#64373=CARTESIAN_POINT('Ctrl Pts',(-21.2077282378307,-18.287564271427,-3.46677656955394));
#64374=CARTESIAN_POINT('Ctrl Pts',(-21.1830026840864,-18.2063554108441,
-3.47099163599204));
#64375=CARTESIAN_POINT('Ctrl Pts',(-21.1585674190593,-18.1260999774808,
-3.47515721572331));
#64376=CARTESIAN_POINT('Ctrl Pts',(-21.1301646741428,-18.0469868800103,
-3.47932279545459));
#64377=CARTESIAN_POINT('Ctrl Pts',(-21.0979289771719,-17.9694320426113,
-3.48348837518587));
#64378=CARTESIAN_POINT('Ctrl Pts',(-21.0657039544922,-17.8919028861496,
-3.48765257555777));
#64379=CARTESIAN_POINT('Ctrl Pts',(-21.0296486772609,-17.815931390789,-3.49181677592968));
#64380=CARTESIAN_POINT('Ctrl Pts',(-20.9899463178963,-17.7419147919381,
-3.49598097630159));
#64381=CARTESIAN_POINT('Ctrl Pts',(-20.9502451090693,-17.6679003380199,
-3.50014505599882));
#64382=CARTESIAN_POINT('Ctrl Pts',(-20.9068972472216,-17.5958410741357,
-3.50430913569606));
#64383=CARTESIAN_POINT('Ctrl Pts',(-20.8601318431732,-17.5261096166098,
-3.50847321539329));
#64384=CARTESIAN_POINT('Ctrl Pts',(-20.8123689128482,-17.4548907569624,
-3.51272611670985));
#64385=CARTESIAN_POINT('Ctrl Pts',(-20.7610412266544,-17.3861005826242,
-3.51697901802641));
#64386=CARTESIAN_POINT('Ctrl Pts',(-20.7064383509254,-17.3201032655836,
-3.52123191934298));
#64387=CARTESIAN_POINT('Ctrl Pts',(-20.6528987388226,-17.2553910923328,
-3.52540200532764));
#64388=CARTESIAN_POINT('Ctrl Pts',(-20.5962107113946,-17.1933642853479,
-3.52957209131231));
#64389=CARTESIAN_POINT('Ctrl Pts',(-20.5366855500211,-17.1343298407728,
-3.53374217729697));
#64390=CARTESIAN_POINT('Ctrl Pts',(-20.4753871892412,-17.0735368147901,
-3.53803648627948));
#64391=CARTESIAN_POINT('Ctrl Pts',(-20.4110803806519,-17.0159176096093,
-3.54233079526199));
#64392=CARTESIAN_POINT('Ctrl Pts',(-20.344141220394,-16.9617625140732,-3.5466251042445));
#64393=CARTESIAN_POINT('Ctrl Pts',(-20.277202060136,-16.9076074185371,-3.55091941322701));
#64394=CARTESIAN_POINT('Ctrl Pts',(-20.2076310154015,-16.8569166856669,
-3.55521372220952));
#64395=CARTESIAN_POINT('Ctrl Pts',(-20.1358342086541,-16.8099307080659,
-3.55950803119203));
#64396=CARTESIAN_POINT('Ctrl Pts',(-20.065871057879,-16.7641447297733,-3.56369266558497));
#64397=CARTESIAN_POINT('Ctrl Pts',(-19.9935321931096,-16.7217048000893,
-3.56787729997791));
#64398=CARTESIAN_POINT('Ctrl Pts',(-19.9191711337668,-16.6828659396841,
-3.57206193437085));
#64399=CARTESIAN_POINT('Ctrl Pts',(-19.844915918188,-16.6440823615894,-3.57624061245468));
#64400=CARTESIAN_POINT('Ctrl Pts',(-19.7686446296087,-16.6088898827212,
-3.58041929053851));
#64401=CARTESIAN_POINT('Ctrl Pts',(-19.6907394622033,-16.5775001365629,
-3.58459796862235));
#64402=CARTESIAN_POINT('Ctrl Pts',(-19.6114379006591,-16.545547751763,-3.58885154650781));
#64403=CARTESIAN_POINT('Ctrl Pts',(-19.5304437130242,-16.5175360325718,
-3.59310512439327));
#64404=CARTESIAN_POINT('Ctrl Pts',(-19.4481859912091,-16.4936390887502,
-3.59735870227874));
#64405=CARTESIAN_POINT('Ctrl Pts',(-19.3675229958468,-16.4702054338166,
-3.60152981625657));
#64406=CARTESIAN_POINT('Ctrl Pts',(-19.2856454833716,-16.4507285663624,
-3.60570093023441));
#64407=CARTESIAN_POINT('Ctrl Pts',(-19.202976239882,-16.4353233647474,-3.60987204421224));
#64408=CARTESIAN_POINT('Ctrl Pts',(-19.1203347368553,-16.4199233324967,
-3.6140417585325));
#64409=CARTESIAN_POINT('Ctrl Pts',(-19.0369024823163,-16.408592336823,-3.61821147285276));
#64410=CARTESIAN_POINT('Ctrl Pts',(-18.9531132034113,-16.4013943064262,
-3.62238118717302));
#64411=CARTESIAN_POINT('Ctrl Pts',(-18.8693269060884,-16.3941965321663,
-3.62655075311694));
#64412=CARTESIAN_POINT('Ctrl Pts',(-18.785184068077,-16.3911314692988,-3.63072031906087));
#64413=CARTESIAN_POINT('Ctrl Pts',(-18.7011229313378,-16.3922111223079,
-3.63488988500479));
#64414=CARTESIAN_POINT('Ctrl Pts',(-18.6141063087262,-16.3933287345849,
-3.63920604774385));
#64415=CARTESIAN_POINT('Ctrl Pts',(-18.5271777668963,-16.398887935209,-3.6435222104829));
#64416=CARTESIAN_POINT('Ctrl Pts',(-18.4408207068908,-16.4088433193977,
-3.64783837322196));
#64417=CARTESIAN_POINT('Ctrl Pts',(-18.3572767190367,-16.418474407993,-3.65201393741352));
#64418=CARTESIAN_POINT('Ctrl Pts',(-18.2742680097319,-16.4322195436239,
-3.65618950160509));
#64419=CARTESIAN_POINT('Ctrl Pts',(-18.1922227301014,-16.4499853338117,
-3.66036506579666));
#64420=CARTESIAN_POINT('Ctrl Pts',(-18.1060335384334,-16.4686484318294,
-3.66475152780946));
#64421=CARTESIAN_POINT('Ctrl Pts',(-18.0209082233736,-16.4917488722623,
-3.66913798982226));
#64422=CARTESIAN_POINT('Ctrl Pts',(-17.9373239039191,-16.5191195676866,
-3.67352445183506));
#64423=CARTESIAN_POINT('Ctrl Pts',(-17.8537395844646,-16.5464902631109,
-3.67791091384786));
#64424=CARTESIAN_POINT('Ctrl Pts',(-17.7716967745984,-16.578130933778,-3.68229737586066));
#64425=CARTESIAN_POINT('Ctrl Pts',(-17.6916449845523,-16.6138177954293,
-3.68668383787345));
#64426=CARTESIAN_POINT('Ctrl Pts',(-17.6152736995718,-16.6478638983293,
-3.6908686254996));
#64427=CARTESIAN_POINT('Ctrl Pts',(-17.5404300949984,-16.6857190326274,
-3.69505341312575));
#64428=CARTESIAN_POINT('Ctrl Pts',(-17.4675200004886,-16.7272239638926,
-3.6992382007519));
#64429=CARTESIAN_POINT('Ctrl Pts',(-17.3947226532098,-16.7686647124668,
-3.70341651707638));
#64430=CARTESIAN_POINT('Ctrl Pts',(-17.3238532703242,-16.813743815844,-3.70759483340085));
#64431=CARTESIAN_POINT('Ctrl Pts',(-17.2552965767961,-16.8622545164051,
-3.71177314972532));
#64432=CARTESIAN_POINT('Ctrl Pts',(-17.2279776972385,-16.8815853492922,
-3.71343815010015));
#64433=CARTESIAN_POINT('Ctrl Pts',(-17.2010258025195,-16.9014605652034,
-3.71510315047499));
#64434=CARTESIAN_POINT('Ctrl Pts',(-17.1744641548914,-16.9218650419685,
-3.71676815084982));
#64435=CARTESIAN_POINT('',(-21.2936055506457,-18.9523823947329,-3.36670986511492));
#64436=CARTESIAN_POINT('Ctrl Pts',(-21.2939999715072,-18.9523819467093,
-3.36670989022851));
#64437=CARTESIAN_POINT('Ctrl Pts',(-21.2940130064034,-18.8650154810554,
-3.3710315430356));
#64438=CARTESIAN_POINT('Ctrl Pts',(-21.2895493128086,-18.777713537132,-3.37535319584269));
#64439=CARTESIAN_POINT('Ctrl Pts',(-21.2806546261691,-18.690944038544,-3.37967484864978));
#64440=CARTESIAN_POINT('Ctrl Pts',(-21.2713805337795,-18.6004733587877,
-3.3841808429622));
#64441=CARTESIAN_POINT('Ctrl Pts',(-21.2572890869443,-18.5105820575898,
-3.38868683727461));
#64442=CARTESIAN_POINT('Ctrl Pts',(-21.2384911684206,-18.4217887333304,
-3.39319283158702));
#64443=CARTESIAN_POINT('Ctrl Pts',(-21.2204017935412,-18.3363422660907,
-3.39752898296562));
#64444=CARTESIAN_POINT('Ctrl Pts',(-21.1979545494933,-18.2519128648075,
-3.40186513434422));
#64445=CARTESIAN_POINT('Ctrl Pts',(-21.1712990035407,-18.1689459997295,
-3.40620128572282));
#64446=CARTESIAN_POINT('Ctrl Pts',(-21.1446099328527,-18.0858747870536,
-3.41054289068799));
#64447=CARTESIAN_POINT('Ctrl Pts',(-21.1137021554184,-18.0042701592823,
-3.41488449565315));
#64448=CARTESIAN_POINT('Ctrl Pts',(-21.078773161122,-17.9245571437388,-3.41922610061831));
#64449=CARTESIAN_POINT('Ctrl Pts',(-21.043770395337,-17.8446757709914,-3.42357687523372));
#64450=CARTESIAN_POINT('Ctrl Pts',(-21.004729634837,-17.7666943545291,-3.42792764984912));
#64451=CARTESIAN_POINT('Ctrl Pts',(-20.9618940508663,-17.6910130460174,
-3.43227842446453));
#64452=CARTESIAN_POINT('Ctrl Pts',(-20.9570751477607,-17.6824990756493,
-3.4327678764426));
#64453=CARTESIAN_POINT('Ctrl Pts',(-20.9522082623988,-17.6740141830165,
-3.43325732842066));
#64454=CARTESIAN_POINT('Ctrl Pts',(-20.9472937739975,-17.6655589131313,
-3.43374678039873));
#64455=CARTESIAN_POINT('Ctrl Pts',(-20.9052767057113,-17.5932694654538,
-3.43793141479118));
#64456=CARTESIAN_POINT('Ctrl Pts',(-20.8596361007271,-17.5229061642046,
-3.44211604918361));
#64457=CARTESIAN_POINT('Ctrl Pts',(-20.8105736599317,-17.4548554395524,
-3.44630068357606));
#64458=CARTESIAN_POINT('Ctrl Pts',(-20.7615810534481,-17.3869015766837,
-3.45047936165939));
#64459=CARTESIAN_POINT('Ctrl Pts',(-20.709176552354,-17.3212541220957,-3.45465803974273));
#64460=CARTESIAN_POINT('Ctrl Pts',(-20.6536069384427,-17.258273575254,-3.45883671782607));
#64461=CARTESIAN_POINT('Ctrl Pts',(-20.597041279129,-17.1941641473619,-3.46309029571166));
#64462=CARTESIAN_POINT('Ctrl Pts',(-20.5371961639064,-17.132818593104,-3.46734387359724));
#64463=CARTESIAN_POINT('Ctrl Pts',(-20.47437711685,-17.0745848910949,-3.47159745148283));
#64464=CARTESIAN_POINT('Ctrl Pts',(-20.4127759396133,-17.0174801630435,
-3.47576856546017));
#64465=CARTESIAN_POINT('Ctrl Pts',(-20.3483154653818,-16.9633680324696,
-3.47993967943751));
#64466=CARTESIAN_POINT('Ctrl Pts',(-20.2813221318917,-16.9125407039713,
-3.48411079341485));
#64467=CARTESIAN_POINT('Ctrl Pts',(-20.2143512786617,-16.8617304310738,
-3.48828050773461));
#64468=CARTESIAN_POINT('Ctrl Pts',(-20.144849620325,-16.8142030489945,-3.49245022205437));
#64469=CARTESIAN_POINT('Ctrl Pts',(-20.0731762130978,-16.7702101223369,
-3.49661993637414));
#64470=CARTESIAN_POINT('Ctrl Pts',(-20.0015053563181,-16.7262187611365,
-3.50078950231757));
#64471=CARTESIAN_POINT('Ctrl Pts',(-19.9276632968148,-16.6857618452166,
-3.504959068261));
#64472=CARTESIAN_POINT('Ctrl Pts',(-19.852036401666,-16.6490465474635,-3.50912863420443));
#64473=CARTESIAN_POINT('Ctrl Pts',(-19.7737505581551,-16.6110403851227,
-3.51344479694407));
#64474=CARTESIAN_POINT('Ctrl Pts',(-19.6935525085948,-16.5770440773061,
-3.51776095968372));
#64475=CARTESIAN_POINT('Ctrl Pts',(-19.6118947218445,-16.5472337208457,
-3.52207712242336));
#64476=CARTESIAN_POINT('Ctrl Pts',(-19.5328969289333,-16.5183944336205,
-3.52625268661445));
#64477=CARTESIAN_POINT('Ctrl Pts',(-19.4525335041398,-16.4934726654687,
-3.53042825080553));
#64478=CARTESIAN_POINT('Ctrl Pts',(-19.3712290384546,-16.4725768508481,
-3.53460381499661));
#64479=CARTESIAN_POINT('Ctrl Pts',(-19.2858180774515,-16.4506256382961,
-3.53899027701054));
#64480=CARTESIAN_POINT('Ctrl Pts',(-19.1993690855433,-16.4331178853207,
-3.54337673902446));
#64481=CARTESIAN_POINT('Ctrl Pts',(-19.1123834602669,-16.4201180997139,
-3.54776320103839));
#64482=CARTESIAN_POINT('Ctrl Pts',(-19.0253978349906,-16.4071183141071,
-3.55214966305231));
#64483=CARTESIAN_POINT('Ctrl Pts',(-18.937876161197,-16.3986264761921,-3.55653612506623));
#64484=CARTESIAN_POINT('Ctrl Pts',(-18.8503205710795,-16.3946440363642,
-3.56092258708016));
#64485=CARTESIAN_POINT('Ctrl Pts',(-18.7668123251306,-16.3908456887752,
-3.5651062805281));
#64486=CARTESIAN_POINT('Ctrl Pts',(-18.68296246577,-16.3911349078501,-3.56928997397603));
#64487=CARTESIAN_POINT('Ctrl Pts',(-18.5992048029022,-16.3955512414994,
-3.57347366742397));
#64488=CARTESIAN_POINT('Ctrl Pts',(-18.5155577245137,-16.3999617443035,
-3.57765183717956));
#64489=CARTESIAN_POINT('Ctrl Pts',(-18.432003055976,-16.4084885197961,-3.58183000693514));
#64490=CARTESIAN_POINT('Ctrl Pts',(-18.3489773389922,-16.4211192144808,
-3.58600817669073));
#64491=CARTESIAN_POINT('Ctrl Pts',(-18.2660363238864,-16.4337370234765,
-3.59018208392577));
#64492=CARTESIAN_POINT('Ctrl Pts',(-18.1836236408616,-16.4504503679989,
-3.59435599116082));
#64493=CARTESIAN_POINT('Ctrl Pts',(-18.1021720696082,-16.4711949963012,
-3.59852989839586));
#64494=CARTESIAN_POINT('Ctrl Pts',(-18.0183963696073,-16.4925315491822,
-3.6028229033677));
#64495=CARTESIAN_POINT('Ctrl Pts',(-17.935637962523,-16.5181329065888,-3.60711590833953));
#64496=CARTESIAN_POINT('Ctrl Pts',(-17.8543574201688,-16.5478725217352,
-3.61140891331137));
#64497=CARTESIAN_POINT('Ctrl Pts',(-17.7754110233124,-16.5767580999032,
-3.61557863541702));
#64498=CARTESIAN_POINT('Ctrl Pts',(-17.6978592079438,-16.6095472799744,
-3.61974835752268));
#64499=CARTESIAN_POINT('Ctrl Pts',(-17.6221076630951,-16.6460738452561,
-3.62391807962833));
#64500=CARTESIAN_POINT('Ctrl Pts',(-17.5429965894828,-16.6842203385134,
-3.62827272603326));
#64501=CARTESIAN_POINT('Ctrl Pts',(-17.4658496781218,-16.7264432229003,
-3.63262737243819));
#64502=CARTESIAN_POINT('Ctrl Pts',(-17.3911026572817,-16.7724985141275,
-3.63698201884312));
#64503=CARTESIAN_POINT('Ctrl Pts',(-17.3163556364417,-16.8185538053548,
-3.64133666524805));
#64504=CARTESIAN_POINT('Ctrl Pts',(-17.2440089783775,-16.8684411823186,
-3.64569131165298));
#64505=CARTESIAN_POINT('Ctrl Pts',(-17.1744641548914,-16.9218650419685,
-3.65004595805791));
#64506=CARTESIAN_POINT('Ctrl Pts',(-17.1767158332876,-16.9247660182631,
-2.85017128494026));
#64507=CARTESIAN_POINT('Ctrl Pts',(-16.7788811275464,-17.2333456901826,
-2.87512870785117));
#64508=CARTESIAN_POINT('Ctrl Pts',(-15.9356499015846,-18.3705873270218,
-2.94247806632256));
#64509=CARTESIAN_POINT('Ctrl Pts',(-16.3642905680513,-20.8355519717216,
-3.05221936035442));
#64510=CARTESIAN_POINT('Ctrl Pts',(-19.0350903593913,-21.9640815770127,
-3.17939516703586));
#64511=CARTESIAN_POINT('Ctrl Pts',(-21.0089153287167,-20.6164715882702,
-3.28422525530707));
#64512=CARTESIAN_POINT('Ctrl Pts',(-21.2903730986671,-19.3569817773889,
-3.34666340801782));
#64513=CARTESIAN_POINT('Ctrl Pts',(-21.2898370719784,-18.9523866753572,
-3.36670962516808));
#64514=CARTESIAN_POINT('Origin',(-18.734,-18.952,1.76670989022851));
#64515=CARTESIAN_POINT('',(-17.1744641548914,-16.9218650419685,-2.05017637359282));
#64516=CARTESIAN_POINT('',(-17.1744641548914,-16.9218650419685,-2.11663751509287));
#64517=CARTESIAN_POINT('',(-17.1744641548914,-16.9218650419685,1.76670989022851));
#64518=CARTESIAN_POINT('',(-21.2939989850553,-18.9497204131755,-2.63329010980608));
#64519=CARTESIAN_POINT('Ctrl Pts',(-17.1744641548914,-16.9218650419685,
-2.11663751509287));
#64520=CARTESIAN_POINT('Ctrl Pts',(-17.1077528165205,-16.9731122376552,
-2.12081218003139));
#64521=CARTESIAN_POINT('Ctrl Pts',(-17.0436083247207,-17.0276217853659,
-2.1249868449699));
#64522=CARTESIAN_POINT('Ctrl Pts',(-16.9823525759525,-17.085095797362,-2.12916150990842));
#64523=CARTESIAN_POINT('Ctrl Pts',(-16.9210594741501,-17.1426048563336,
-2.13333872050844));
#64524=CARTESIAN_POINT('Ctrl Pts',(-16.8626589411317,-17.2030816470779,
-2.13751593110846));
#64525=CARTESIAN_POINT('Ctrl Pts',(-16.8074345510184,-17.2661929022601,
-2.14169314170848));
#64526=CARTESIAN_POINT('Ctrl Pts',(-16.7521184201283,-17.3294090001678,
-2.14587729164354));
#64527=CARTESIAN_POINT('Ctrl Pts',(-16.6999892500854,-17.3952679385715,
-2.15006144157861));
#64528=CARTESIAN_POINT('Ctrl Pts',(-16.6512887918949,-17.4634053528132,
-2.15424559151367));
#64529=CARTESIAN_POINT('Ctrl Pts',(-16.6267354913389,-17.4977581797299,
-2.15635511357453));
#64530=CARTESIAN_POINT('Ctrl Pts',(-16.6030530181617,-17.5326897371648,
-2.15846463563539));
#64531=CARTESIAN_POINT('Ctrl Pts',(-16.5802679097402,-17.5681509896722,
-2.16057415769624));
#64532=CARTESIAN_POINT('Ctrl Pts',(-16.5350693576943,-17.6384950599053,
-2.16475879183957));
#64533=CARTESIAN_POINT('Ctrl Pts',(-16.493236628805,-17.7111867434462,-2.1689434259829));
#64534=CARTESIAN_POINT('Ctrl Pts',(-16.4550217747166,-17.78587039799,-2.17312806012622));
#64535=CARTESIAN_POINT('Ctrl Pts',(-16.4168613147862,-17.860447749511,-2.17730673795607));
#64536=CARTESIAN_POINT('Ctrl Pts',(-16.3823087086902,-17.9370110341541,
-2.18148541578591));
#64537=CARTESIAN_POINT('Ctrl Pts',(-16.3515723823109,-18.015176299151,-2.18566409361575));
#64538=CARTESIAN_POINT('Ctrl Pts',(-16.3202851270053,-18.094742626363,-2.18991767156416));
#64539=CARTESIAN_POINT('Ctrl Pts',(-16.2929525719636,-18.17596852444,-2.19417124951258));
#64540=CARTESIAN_POINT('Ctrl Pts',(-16.2697452280173,-18.2584234586145,
-2.19842482746099));
#64541=CARTESIAN_POINT('Ctrl Pts',(-16.2469878054909,-18.3392798366959,
-2.20259594117589));
#64542=CARTESIAN_POINT('Ctrl Pts',(-16.2281972006544,-18.4213175582041,
-2.20676705489078));
#64543=CARTESIAN_POINT('Ctrl Pts',(-16.2134847477736,-18.5041128900111,
-2.21093816860568));
#64544=CARTESIAN_POINT('Ctrl Pts',(-16.1987772318086,-18.5868804389882,
-2.21510788266023));
#64545=CARTESIAN_POINT('Ctrl Pts',(-16.1881452304225,-18.6704046408108,
-2.21927759671478));
#64546=CARTESIAN_POINT('Ctrl Pts',(-16.1816490383963,-18.7542512482957,
-2.22344731076934));
#64547=CARTESIAN_POINT('Ctrl Pts',(-16.1751530775363,-18.8380948721096,
-2.22761687644513));
#64548=CARTESIAN_POINT('Ctrl Pts',(-16.1727926681059,-18.9222604200508,
-2.23178644212093));
#64549=CARTESIAN_POINT('Ctrl Pts',(-16.1745761446872,-19.0063095650504,
-2.23595600779672));
#64550=CARTESIAN_POINT('Ctrl Pts',(-16.1764223263562,-19.0933137861386,
-2.24027217084513));
#64551=CARTESIAN_POINT('Ctrl Pts',(-16.1827092038591,-19.1801927391925,
-2.24458833389355));
#64552=CARTESIAN_POINT('Ctrl Pts',(-16.1933873263743,-19.2664634201504,
-2.24890449694196));
#64553=CARTESIAN_POINT('Ctrl Pts',(-16.2037176087591,-19.3499238313372,
-2.25308006086206));
#64554=CARTESIAN_POINT('Ctrl Pts',(-16.218157311486,-19.4328145349869,-2.25725562478215));
#64555=CARTESIAN_POINT('Ctrl Pts',(-16.2366094603544,-19.5147081770233,
-2.26143118870225));
#64556=CARTESIAN_POINT('Ctrl Pts',(-16.2559935873087,-19.600738089599,-2.26581765131482));
#64557=CARTESIAN_POINT('Ctrl Pts',(-16.2798059943325,-19.6856670076962,
-2.27020411392739));
#64558=CARTESIAN_POINT('Ctrl Pts',(-16.3078756047366,-19.7690192278692,
-2.27459057653996));
#64559=CARTESIAN_POINT('Ctrl Pts',(-16.3359452151407,-19.8523714480422,
-2.27897703915254));
#64560=CARTESIAN_POINT('Ctrl Pts',(-16.3682717448824,-19.9341464586679,
-2.28336350176511));
#64561=CARTESIAN_POINT('Ctrl Pts',(-16.4046276535555,-20.0138966388589,
-2.28774996437768));
#64562=CARTESIAN_POINT('Ctrl Pts',(-16.4393107693605,-20.0899773871051,
-2.29193459890665));
#64563=CARTESIAN_POINT('Ctrl Pts',(-16.4777897133297,-20.1644987286687,
-2.29611923343562));
#64564=CARTESIAN_POINT('Ctrl Pts',(-16.5199018772369,-20.2370562255314,
-2.30030386796459));
#64565=CARTESIAN_POINT('Ctrl Pts',(-16.5619540997103,-20.3095104458109,
-2.30448254618615));
#64566=CARTESIAN_POINT('Ctrl Pts',(-16.6076290410699,-20.380005979242,-2.30866122440772));
#64567=CARTESIAN_POINT('Ctrl Pts',(-16.6567166746768,-20.4481597462618,
-2.31283990262929));
#64568=CARTESIAN_POINT('Ctrl Pts',(-16.7066841667901,-20.5175351177317,
-2.31709348048053));
#64569=CARTESIAN_POINT('Ctrl Pts',(-16.7601876992645,-20.5844835062087,
-2.32134705833178));
#64570=CARTESIAN_POINT('Ctrl Pts',(-16.8169575547711,-20.6486284988738,
-2.32560063618302));
#64571=CARTESIAN_POINT('Ctrl Pts',(-16.8726268181782,-20.7115299183165,
-2.32977175030178));
#64572=CARTESIAN_POINT('Ctrl Pts',(-16.931436568049,-20.7717353099527,-2.33394286442054));
#64573=CARTESIAN_POINT('Ctrl Pts',(-16.9930907749213,-20.8289217005608,
-2.3381139785393));
#64574=CARTESIAN_POINT('Ctrl Pts',(-17.0547242931429,-20.8860889017359,
-2.34228369300136));
#64575=CARTESIAN_POINT('Ctrl Pts',(-17.1192000357421,-20.9402388012432,
-2.34645340746342));
#64576=CARTESIAN_POINT('Ctrl Pts',(-17.1861855059002,-20.9910856509364,
-2.35062312192549));
#64577=CARTESIAN_POINT('Ctrl Pts',(-17.253168592439,-21.041930691289,-2.35479268801191));
#64578=CARTESIAN_POINT('Ctrl Pts',(-17.3226608620329,-21.0894726380556,
-2.35896225409833));
#64579=CARTESIAN_POINT('Ctrl Pts',(-17.3942982622585,-21.1334672250329,
-2.36313182018476));
#64580=CARTESIAN_POINT('Ctrl Pts',(-17.4684543397166,-21.1790086041077,
-2.36744798275762));
#64581=CARTESIAN_POINT('Ctrl Pts',(-17.5449087502468,-21.2207482563335,
-2.37176414533048));
#64582=CARTESIAN_POINT('Ctrl Pts',(-17.6232285972719,-21.2584663212112,
-2.37608030790335));
#64583=CARTESIAN_POINT('Ctrl Pts',(-17.6989971890216,-21.2949557267432,
-2.38025587223768));
#64584=CARTESIAN_POINT('Ctrl Pts',(-17.7765110983774,-21.3276813875021,
-2.38443143657202));
#64585=CARTESIAN_POINT('Ctrl Pts',(-17.8553584978293,-21.3564935247705,
-2.38860700090636));
#64586=CARTESIAN_POINT('Ctrl Pts',(-17.9381882831052,-21.3867608913529,
-2.39299346259849));
#64587=CARTESIAN_POINT('Ctrl Pts',(-18.0224892495074,-21.4127088296275,
-2.39737992429061));
#64588=CARTESIAN_POINT('Ctrl Pts',(-18.1077688055337,-21.4342236988389,
-2.40176638598274));
#64589=CARTESIAN_POINT('Ctrl Pts',(-18.1930483615599,-21.4557385680502,
-2.40615284767487));
#64590=CARTESIAN_POINT('Ctrl Pts',(-18.2793059232703,-21.4728203301016,
-2.41053930936699));
#64591=CARTESIAN_POINT('Ctrl Pts',(-18.3660419494156,-21.4854180217663,
-2.41492577105912));
#64592=CARTESIAN_POINT('Ctrl Pts',(-18.4487871282886,-21.4974360758149,
-2.41911040544306));
#64593=CARTESIAN_POINT('Ctrl Pts',(-18.5322757027619,-21.5054183621378,
-2.42329503982701));
#64594=CARTESIAN_POINT('Ctrl Pts',(-18.6160795877487,-21.5092826938715,
-2.42747967421095));
#64595=CARTESIAN_POINT('Ctrl Pts',(-18.6997641882823,-21.5131415252074,
-2.43165835228601));
#64596=CARTESIAN_POINT('Ctrl Pts',(-18.7837627522466,-21.5128940235268,
-2.43583703036108));
#64597=CARTESIAN_POINT('Ctrl Pts',(-18.867639486945,-21.5085094342734,-2.44001570843614));
#64598=CARTESIAN_POINT('Ctrl Pts',(-18.9530196520584,-21.504046254397,-2.44426928632383));
#64599=CARTESIAN_POINT('Ctrl Pts',(-19.0382731002339,-21.4952961442205,
-2.44852286421151));
#64600=CARTESIAN_POINT('Ctrl Pts',(-19.1229373349508,-21.4822821481964,
-2.45277644209919));
#64601=CARTESIAN_POINT('Ctrl Pts',(-19.2059601880607,-21.469520453912,-2.45694755606889));
#64602=CARTESIAN_POINT('Ctrl Pts',(-19.2884159943129,-21.4526587990527,
-2.46111867003858));
#64603=CARTESIAN_POINT('Ctrl Pts',(-19.3698729492297,-21.4317712782509,
-2.46528978400827));
#64604=CARTESIAN_POINT('Ctrl Pts',(-19.4513025704834,-21.4108907664571,
-2.46945949832063));
#64605=CARTESIAN_POINT('Ctrl Pts',(-19.531733560818,-21.3859871858369,-2.47362921263299));
#64606=CARTESIAN_POINT('Ctrl Pts',(-19.6107456770632,-21.3571854435264,
-2.47779892694536));
#64607=CARTESIAN_POINT('Ctrl Pts',(-19.6897549817234,-21.3283847261035,
-2.48196849288167));
#64608=CARTESIAN_POINT('Ctrl Pts',(-19.7673450807596,-21.2956862811396,
-2.48613805881798));
#64609=CARTESIAN_POINT('Ctrl Pts',(-19.8431135302991,-21.2592640024296,
-2.4903076247543));
#64610=CARTESIAN_POINT('Ctrl Pts',(-19.9215459053798,-21.2215611611752,
-2.49462378750315));
#64611=CARTESIAN_POINT('Ctrl Pts',(-19.9980256738089,-21.1798679825043,
-2.498939950252));
#64612=CARTESIAN_POINT('Ctrl Pts',(-20.0721336489201,-21.1344294576522,
-2.50325611300086));
#64613=CARTESIAN_POINT('Ctrl Pts',(-20.1438275642515,-21.0904710881427,
-2.50743167718554));
#64614=CARTESIAN_POINT('Ctrl Pts',(-20.2133014733422,-21.0430079392836,
-2.51160724137021));
#64615=CARTESIAN_POINT('Ctrl Pts',(-20.2802065215954,-20.9923052204452,
-2.51578280555489));
#64616=CARTESIAN_POINT('Ctrl Pts',(-20.3504907851969,-20.9390416274998,
-2.52016926758584));
#64617=CARTESIAN_POINT('Ctrl Pts',(-20.4179394151663,-20.8822029788412,
-2.52455572961678));
#64618=CARTESIAN_POINT('Ctrl Pts',(-20.482190227081,-20.8221419544886,-2.52894219164772));
#64619=CARTESIAN_POINT('Ctrl Pts',(-20.5464410389958,-20.7620809301359,
-2.53332865367867));
#64620=CARTESIAN_POINT('Ctrl Pts',(-20.6074936847468,-20.6987980004696,
-2.53771511570961));
#64621=CARTESIAN_POINT('Ctrl Pts',(-20.6650349200516,-20.6326856153193,
-2.54210157774055));
#64622=CARTESIAN_POINT('Ctrl Pts',(-20.7194682477086,-20.5701440813393,
-2.54625111891256));
#64623=CARTESIAN_POINT('Ctrl Pts',(-20.7709705307815,-20.5048282635486,
-2.55040066008456));
#64624=CARTESIAN_POINT('Ctrl Pts',(-20.8192426277936,-20.4370465256121,
-2.55455020125656));
#64625=CARTESIAN_POINT('Ctrl Pts',(-20.8674506257188,-20.3693547930364,
-2.55869423237583));
#64626=CARTESIAN_POINT('Ctrl Pts',(-20.9124366796727,-20.2992040148273,
-2.5628382634951));
#64627=CARTESIAN_POINT('Ctrl Pts',(-20.9539402798274,-20.226937313753,-2.56698229461437));
#64628=CARTESIAN_POINT('Ctrl Pts',(-20.9954017278076,-20.1547440086875,
-2.57112211694398));
#64629=CARTESIAN_POINT('Ctrl Pts',(-21.0333875106771,-20.0804394498645,
-2.57526193927359));
#64630=CARTESIAN_POINT('Ctrl Pts',(-21.0676798966755,-20.0043963796272,
-2.5794017616032));
#64631=CARTESIAN_POINT('Ctrl Pts',(-21.1019481578627,-19.9284068059507,
-2.5835386715536));
#64632=CARTESIAN_POINT('Ctrl Pts',(-21.1325279904582,-19.8506815753028,
-2.58767558150399));
#64633=CARTESIAN_POINT('Ctrl Pts',(-21.1592478841602,-19.771617410977,-2.59181249145439));
#64634=CARTESIAN_POINT('Ctrl Pts',(-21.185962767488,-19.6925680723481,-2.59594862567316));
#64635=CARTESIAN_POINT('Ctrl Pts',(-21.2088189905539,-19.6121807387845,
-2.60008475989194));
#64636=CARTESIAN_POINT('Ctrl Pts',(-21.2276938748169,-19.5308703297809,
-2.60422089411071));
#64637=CARTESIAN_POINT('Ctrl Pts',(-21.2465668271854,-19.4495682431134,
-2.60835660498518));
#64638=CARTESIAN_POINT('Ctrl Pts',(-21.2614591515706,-19.3673437264561,
-2.61249231585964));
#64639=CARTESIAN_POINT('Ctrl Pts',(-21.2722989879432,-19.2846232821176,
-2.61662802673411));
#64640=CARTESIAN_POINT('Ctrl Pts',(-21.2831447249165,-19.2018578093952,
-2.62076598885829));
#64641=CARTESIAN_POINT('Ctrl Pts',(-21.2899335186421,-19.1185963356274,
-2.62490395098247));
#64642=CARTESIAN_POINT('Ctrl Pts',(-21.2926453380223,-19.0352708485401,
-2.62904191310665));
#64643=CARTESIAN_POINT('Ctrl Pts',(-21.2935733586036,-19.0067557610229,
-2.6304579786616));
#64644=CARTESIAN_POINT('Ctrl Pts',(-21.2940243746442,-18.9782331861905,
-2.63187404421655));
#64645=CARTESIAN_POINT('Ctrl Pts',(-21.2939989850559,-18.9497204138719,
-2.6332901097715));
#64646=CARTESIAN_POINT('Ctrl Pts',(-21.2939989850553,-18.9497204131756,
-2.63329010980608));
#64647=CARTESIAN_POINT('Ctrl Pts',(-21.2939071256071,-18.8465613267959,
-2.63841342883209));
#64648=CARTESIAN_POINT('Ctrl Pts',(-21.287576105512,-18.7436786900576,-2.6435367478581));
#64649=CARTESIAN_POINT('Ctrl Pts',(-21.275128076311,-18.6417289897787,-2.64866006688411));
#64650=CARTESIAN_POINT('Ctrl Pts',(-21.262474961387,-18.538099631808,-2.65386779441926));
#64651=CARTESIAN_POINT('Ctrl Pts',(-21.243501668497,-18.4354341184935,-2.65907552195442));
#64652=CARTESIAN_POINT('Ctrl Pts',(-21.2183850428296,-18.3343990293364,
-2.66428324948958));
#64653=CARTESIAN_POINT('Ctrl Pts',(-21.2103562166424,-18.3021019691982,
-2.66594796113372));
#64654=CARTESIAN_POINT('Ctrl Pts',(-21.2017000060005,-18.2699713447231,
-2.66761267277785));
#64655=CARTESIAN_POINT('Ctrl Pts',(-21.1924232051049,-18.2380284707345,
-2.66927738442199));
#64656=CARTESIAN_POINT('Ctrl Pts',(-21.1691038390101,-18.1577327328991,
-2.67346201883518));
#64657=CARTESIAN_POINT('Ctrl Pts',(-21.1418030734485,-18.078431236944,-2.67764665324838));
#64658=CARTESIAN_POINT('Ctrl Pts',(-21.1106233366666,-18.0005476808522,
-2.68183128766158));
#64659=CARTESIAN_POINT('Ctrl Pts',(-21.0794879803785,-17.922774982357,-2.68600996576594));
#64660=CARTESIAN_POINT('Ctrl Pts',(-21.0444847892945,-17.8464166382494,
-2.69018864387031));
#64661=CARTESIAN_POINT('Ctrl Pts',(-21.0057661997858,-17.7718820679649,
-2.69436732197467));
#64662=CARTESIAN_POINT('Ctrl Pts',(-20.9663536076263,-17.6960115195364,
-2.69862089985503));
#64663=CARTESIAN_POINT('Ctrl Pts',(-20.923091244402,-17.6220312333054,-2.7028744777354));
#64664=CARTESIAN_POINT('Ctrl Pts',(-20.8761915739221,-17.5503526618235,
-2.70712805561576));
#64665=CARTESIAN_POINT('Ctrl Pts',(-20.8302011447859,-17.4800637188825,
-2.71129916961464));
#64666=CARTESIAN_POINT('Ctrl Pts',(-20.7807134458741,-17.4119884433551,
-2.71547028361352));
#64667=CARTESIAN_POINT('Ctrl Pts',(-20.727974702693,-17.3464892136705,-2.7196413976124));
#64668=CARTESIAN_POINT('Ctrl Pts',(-20.6752536565046,-17.2810119628826,
-2.72381111195385));
#64669=CARTESIAN_POINT('Ctrl Pts',(-20.6192840209005,-17.2181093992114,
-2.7279808262953));
#64670=CARTESIAN_POINT('Ctrl Pts',(-20.560353487424,-17.1581123393662,-2.73215054063674));
#64671=CARTESIAN_POINT('Ctrl Pts',(-20.5014250509472,-17.0981174144723,
-2.73632010660198));
#64672=CARTESIAN_POINT('Ctrl Pts',(-20.4395362490537,-17.0410281154373,
-2.74048967256722));
#64673=CARTESIAN_POINT('Ctrl Pts',(-20.3750119946106,-16.987138774991,-2.74465923853245));
#64674=CARTESIAN_POINT('Ctrl Pts',(-20.308219147702,-16.9313547524166,-2.7489754012467));
#64675=CARTESIAN_POINT('Ctrl Pts',(-20.2386024799444,-16.8790002342649,
-2.75329156396095));
#64676=CARTESIAN_POINT('Ctrl Pts',(-20.1665585535975,-16.8303553571546,
-2.75760772667519));
#64677=CARTESIAN_POINT('Ctrl Pts',(-20.0968614498202,-16.7832950812909,
-2.76178329088814));
#64678=CARTESIAN_POINT('Ctrl Pts',(-20.0248932222052,-16.7397066785479,
-2.76595885510109));
#64679=CARTESIAN_POINT('Ctrl Pts',(-19.9510397172924,-16.6997978939418,
-2.77013441931403));
#64680=CARTESIAN_POINT('Ctrl Pts',(-19.8734560486543,-16.6578734121683,
-2.77452088127893));
#64681=CARTESIAN_POINT('Ctrl Pts',(-19.7937921742853,-16.6200102829178,
-2.77890734324383));
#64682=CARTESIAN_POINT('Ctrl Pts',(-19.7125190809675,-16.5863921694029,
-2.78329380520873));
#64683=CARTESIAN_POINT('Ctrl Pts',(-19.6312459876497,-16.552774055888,-2.78768026717362));
#64684=CARTESIAN_POINT('Ctrl Pts',(-19.5483642476805,-16.5234010802283,
-2.79206672913852));
#64685=CARTESIAN_POINT('Ctrl Pts',(-19.464360786173,-16.4983958913426,-2.79645319110342));
#64686=CARTESIAN_POINT('Ctrl Pts',(-19.3842194543361,-16.4745403370097,
-2.80063798179669));
#64687=CARTESIAN_POINT('Ctrl Pts',(-19.3027589678988,-16.4545709643748,
-2.80482277248996));
#64688=CARTESIAN_POINT('Ctrl Pts',(-19.2203910787736,-16.4386310023219,
-2.80900756318323));
#64689=CARTESIAN_POINT('Ctrl Pts',(-19.138141261341,-16.4227138896867,-2.81318635511502));
#64690=CARTESIAN_POINT('Ctrl Pts',(-19.0549870728687,-16.4108148007743,
-2.81736514704681));
#64691=CARTESIAN_POINT('Ctrl Pts',(-18.9713553167887,-16.4030271767647,
-2.82154393897861));
#64692=CARTESIAN_POINT('Ctrl Pts',(-18.8878237953098,-16.3952488864033,
-2.82571772253126));
#64693=CARTESIAN_POINT('Ctrl Pts',(-18.8038162997764,-16.3915723068654,
-2.82989150608392));
#64694=CARTESIAN_POINT('Ctrl Pts',(-18.7197682827838,-16.3920395592461,
-2.83406528963658));
#64695=CARTESIAN_POINT('Ctrl Pts',(-18.6357753750601,-16.392506505255,-2.8382363364898));
#64696=CARTESIAN_POINT('Ctrl Pts',(-18.5517424573058,-16.3971118856058,
-2.84240738334303));
#64697=CARTESIAN_POINT('Ctrl Pts',(-18.4681074911956,-16.4058458071512,
-2.84657843019625));
#64698=CARTESIAN_POINT('Ctrl Pts',(-18.3845022745217,-16.4145766219907,
-2.85074799338423));
#64699=CARTESIAN_POINT('Ctrl Pts',(-18.3012951853525,-16.4274330128497,
-2.85491755657221));
#64700=CARTESIAN_POINT('Ctrl Pts',(-18.2189201971835,-16.444353135561,-2.85908711976019));
#64701=CARTESIAN_POINT('Ctrl Pts',(-18.1365498000672,-16.4612723152535,
-2.8632564505635));
#64702=CARTESIAN_POINT('Ctrl Pts',(-18.055011861932,-16.4822546823771,-2.86742578136681));
#64703=CARTESIAN_POINT('Ctrl Pts',(-17.9747299315152,-16.5071873357856,
-2.87159511217012));
#64704=CARTESIAN_POINT('Ctrl Pts',(-17.894383666535,-16.5321399691742,-2.87576778409983));
#64705=CARTESIAN_POINT('Ctrl Pts',(-17.8152958594281,-16.5610490742598,
-2.87994045602953));
#64706=CARTESIAN_POINT('Ctrl Pts',(-17.7378740400419,-16.5937521182247,
-2.88411312795923));
#64707=CARTESIAN_POINT('Ctrl Pts',(-17.6604189341378,-16.6264692224438,
-2.8882875938757));
#64708=CARTESIAN_POINT('Ctrl Pts',(-17.5846316580742,-16.6629833163545,
-2.89246205979216));
#64709=CARTESIAN_POINT('Ctrl Pts',(-17.5108968677673,-16.7030849887285,
-2.89663652570862));
#64710=CARTESIAN_POINT('Ctrl Pts',(-17.4370550940829,-16.7432448454728,
-2.90081704844658));
#64711=CARTESIAN_POINT('Ctrl Pts',(-17.3652721468036,-16.7870024370522,
-2.90499757118454));
#64712=CARTESIAN_POINT('Ctrl Pts',(-17.2959049510485,-16.8341041975156,
-2.9091780939225));
#64713=CARTESIAN_POINT('Ctrl Pts',(-17.2545430745508,-16.8621897670402,
-2.91167083221616));
#64714=CARTESIAN_POINT('Ctrl Pts',(-17.2140395108878,-16.8914635230867,
-2.91416357050983));
#64715=CARTESIAN_POINT('Ctrl Pts',(-17.1744641548914,-16.9218650419685,
-2.9166563088035));
#64716=CARTESIAN_POINT('',(-21.2939990581247,-18.9541959965425,-2.56670989022851));
#64717=CARTESIAN_POINT('Ctrl Pts',(-21.2953147714723,-18.9541844553181,
-2.56671052139392));
#64718=CARTESIAN_POINT('Ctrl Pts',(-21.288986792687,-18.2584132339351,-2.60137099436598));
#64719=CARTESIAN_POINT('Ctrl Pts',(-20.6359183782719,-16.7012242333178,
-2.67842340289853));
#64720=CARTESIAN_POINT('Ctrl Pts',(-18.5512406649392,-16.1584580776078,
-2.77291032408065));
#64721=CARTESIAN_POINT('Ctrl Pts',(-17.4546313149639,-16.7092014460441,
-2.8327367722907));
#64722=CARTESIAN_POINT('Ctrl Pts',(-17.1767158332876,-16.9247660182631,
-2.85017128494026));
#64723=CARTESIAN_POINT('Ctrl Pts',(-17.1744641548914,-16.9218650419685,
-2.05017637359282));
#64724=CARTESIAN_POINT('Ctrl Pts',(-17.1080052683081,-16.9729183059117,
-2.05435390665174));
#64725=CARTESIAN_POINT('Ctrl Pts',(-17.0439627308144,-17.0273100309957,
-2.05853143971067));
#64726=CARTESIAN_POINT('Ctrl Pts',(-16.9826883158293,-17.0847808417631,
-2.06270897276959));
#64727=CARTESIAN_POINT('Ctrl Pts',(-16.9214786472874,-17.1421909252172,
-2.06688209158143));
#64728=CARTESIAN_POINT('Ctrl Pts',(-16.8630316217416,-17.2026733145463,
-2.07105521039328));
#64729=CARTESIAN_POINT('Ctrl Pts',(-16.8076661469867,-17.2659282676188,
-2.07522832920512));
#64730=CARTESIAN_POINT('Ctrl Pts',(-16.7523324560721,-17.3291469077122,
-2.07939905234092));
#64731=CARTESIAN_POINT('Ctrl Pts',(-16.700077106004,-17.3951346061225,-2.08356977547672));
#64732=CARTESIAN_POINT('Ctrl Pts',(-16.6511815089029,-17.4635554652107,
-2.08774049861252));
#64733=CARTESIAN_POINT('Ctrl Pts',(-16.6022993137412,-17.5319575706226,
-2.09191007858244));
#64734=CARTESIAN_POINT('Ctrl Pts',(-16.5567753097313,-17.6027911379656,
-2.09607965855236));
#64735=CARTESIAN_POINT('Ctrl Pts',(-16.5148491823605,-17.6756890470696,
-2.10024923852227));
#64736=CARTESIAN_POINT('Ctrl Pts',(-16.4729219698532,-17.7485888429253,
-2.10441892640972));
#64737=CARTESIAN_POINT('Ctrl Pts',(-16.434593047127,-17.8235526871958,-2.10858861429716));
#64738=CARTESIAN_POINT('Ctrl Pts',(-16.4000568074652,-17.9001876716732,
-2.11275830218461));
#64739=CARTESIAN_POINT('Ctrl Pts',(-16.3654854752132,-17.9769005256618,
-2.11693222693019));
#64740=CARTESIAN_POINT('Ctrl Pts',(-16.3347147131887,-18.0552874912678,
-2.12110615167577));
#64741=CARTESIAN_POINT('Ctrl Pts',(-16.307891067568,-18.1349348569584,-2.12528007642135));
#64742=CARTESIAN_POINT('Ctrl Pts',(-16.2810541182091,-18.2146217253965,
-2.12945607131067));
#64743=CARTESIAN_POINT('Ctrl Pts',(-16.2581683100149,-18.2955697959418,
-2.13363206619998));
#64744=CARTESIAN_POINT('Ctrl Pts',(-16.239329813502,-18.3773517070432,-2.13780806108929));
#64745=CARTESIAN_POINT('Ctrl Pts',(-16.2204575476003,-18.4592802182279,
-2.14199154175622));
#64746=CARTESIAN_POINT('Ctrl Pts',(-16.205647171031,-18.542045102734,-2.14617502242315));
#64747=CARTESIAN_POINT('Ctrl Pts',(-16.1949433667954,-18.6252104448122,
-2.15035850309007));
#64748=CARTESIAN_POINT('Ctrl Pts',(-16.1850243937153,-18.7022778846793,
-2.15423523992151));
#64749=CARTESIAN_POINT('Ctrl Pts',(-16.1786313142725,-18.7796888613376,
-2.15811197675294));
#64750=CARTESIAN_POINT('Ctrl Pts',(-16.1757597065435,-18.8570968865864,
-2.16198871358438));
#64751=CARTESIAN_POINT('Ctrl Pts',(-16.172660029791,-18.9406528172576,-2.16617334887092));
#64752=CARTESIAN_POINT('Ctrl Pts',(-16.1736524807757,-19.0245162611934,
-2.17035798415747));
#64753=CARTESIAN_POINT('Ctrl Pts',(-16.1787729919005,-19.1082527986266,
-2.17454261944402));
#64754=CARTESIAN_POINT('Ctrl Pts',(-16.1838862146257,-19.1918701476969,
-2.17872129843186));
#64755=CARTESIAN_POINT('Ctrl Pts',(-16.1931157985219,-19.2753604938156,
-2.18289997741971));
#64756=CARTESIAN_POINT('Ctrl Pts',(-16.2064457143536,-19.3582872544277,
-2.18707865640756));
#64757=CARTESIAN_POINT('Ctrl Pts',(-16.2200145556947,-19.4427003949071,
-2.19133223406832));
#64758=CARTESIAN_POINT('Ctrl Pts',(-16.2378321873097,-19.5265290651159,
-2.19558581172908));
#64759=CARTESIAN_POINT('Ctrl Pts',(-16.2598262336471,-19.6093158859262,
-2.19983938938984));
#64760=CARTESIAN_POINT('Ctrl Pts',(-16.2813938883893,-19.6904977449191,
-2.20401050429063));
#64761=CARTESIAN_POINT('Ctrl Pts',(-16.3069773456877,-19.7706773249541,
-2.20818161919142));
#64762=CARTESIAN_POINT('Ctrl Pts',(-16.3364567550223,-19.8494332222854,
-2.21235273409221));
#64763=CARTESIAN_POINT('Ctrl Pts',(-16.3659262722942,-19.9281626924159,
-2.21652244934048));
#64764=CARTESIAN_POINT('Ctrl Pts',(-16.3992889841105,-20.0054689981388,
-2.22069216458874));
#64765=CARTESIAN_POINT('Ctrl Pts',(-16.4363757553429,-20.0809476650243,
-2.224861879837));
#64766=CARTESIAN_POINT('Ctrl Pts',(-16.4734612069031,-20.1564236461247,
-2.22903144671276));
#64767=CARTESIAN_POINT('Ctrl Pts',(-16.5142702507692,-20.2300717051833,
-2.23320101358851));
#64768=CARTESIAN_POINT('Ctrl Pts',(-16.5585869497193,-20.3015103040246,
-2.23737058046427));
#64769=CARTESIAN_POINT('Ctrl Pts',(-16.6044617473107,-20.3754605606929,
-2.2416867421144));
#64770=CARTESIAN_POINT('Ctrl Pts',(-16.6540951659904,-20.4470426511764,
-2.24600290376453));
#64771=CARTESIAN_POINT('Ctrl Pts',(-16.7071987886738,-20.515865994824,-2.25031906541466));
#64772=CARTESIAN_POINT('Ctrl Pts',(-16.758572590857,-20.5824474569441,-2.25449463053808));
#64773=CARTESIAN_POINT('Ctrl Pts',(-16.8131936465655,-20.646446814372,-2.25867019566151));
#64774=CARTESIAN_POINT('Ctrl Pts',(-16.8707609580349,-20.7075455768783,
-2.26284576078493));
#64775=CARTESIAN_POINT('Ctrl Pts',(-16.9312358151196,-20.7717302475935,
-2.26723222069841));
#64776=CARTESIAN_POINT('Ctrl Pts',(-16.994961954188,-20.8327132054428,-2.27161868061189));
#64777=CARTESIAN_POINT('Ctrl Pts',(-17.0615499837251,-20.8901720622953,
-2.27600514052537));
#64778=CARTESIAN_POINT('Ctrl Pts',(-17.1281380132622,-20.9476309191478,
-2.28039160043886));
#64779=CARTESIAN_POINT('Ctrl Pts',(-17.1975874283579,-21.0015653791984,
-2.28477806035234));
#64780=CARTESIAN_POINT('Ctrl Pts',(-17.2694745299266,-21.0517059669168,
-2.28916452026582));
#64781=CARTESIAN_POINT('Ctrl Pts',(-17.3380540324737,-21.0995395349439,
-2.29334915467512));
#64782=CARTESIAN_POINT('Ctrl Pts',(-17.4091070955212,-21.1440987240517,
-2.29753378908443));
#64783=CARTESIAN_POINT('Ctrl Pts',(-17.4822878905414,-21.1851181775792,
-2.30171842349373));
#64784=CARTESIAN_POINT('Ctrl Pts',(-17.5553645218076,-21.2260792450197,
-2.30589710159675));
#64785=CARTESIAN_POINT('Ctrl Pts',(-17.6305624715103,-21.2635103616649,
-2.31007577969977));
#64786=CARTESIAN_POINT('Ctrl Pts',(-17.7075059666942,-21.2971886916808,
-2.31425445780279));
#64787=CARTESIAN_POINT('Ctrl Pts',(-17.7858286182921,-21.331470681366,-2.31850803568381));
#64788=CARTESIAN_POINT('Ctrl Pts',(-17.8659596132195,-21.3618637479389,
-2.32276161356483));
#64789=CARTESIAN_POINT('Ctrl Pts',(-17.947475192358,-21.3881811769579,-2.32701519144585));
#64790=CARTESIAN_POINT('Ctrl Pts',(-18.0274104335102,-21.4139883914482,
-2.33118630544973));
#64791=CARTESIAN_POINT('Ctrl Pts',(-18.1086765942978,-21.4358764386359,
-2.33535741945361));
#64792=CARTESIAN_POINT('Ctrl Pts',(-18.1908544682179,-21.453717995959,-2.33952853345749));
#64793=CARTESIAN_POINT('Ctrl Pts',(-18.2730047666085,-21.471553566386,-2.3436982478063));
#64794=CARTESIAN_POINT('Ctrl Pts',(-18.3560657213573,-21.4853452461106,
-2.3478679621551));
#64795=CARTESIAN_POINT('Ctrl Pts',(-18.4396056840043,-21.4950163166424,
-2.35203767650391));
#64796=CARTESIAN_POINT('Ctrl Pts',(-18.5231426739907,-21.5046870430418,
-2.35620724247888));
#64797=CARTESIAN_POINT('Ctrl Pts',(-18.6071581809069,-21.5102373997233,
-2.36037680845384));
#64798=CARTESIAN_POINT('Ctrl Pts',(-18.6912145089616,-21.5116424363095,
-2.36454637442881));
#64799=CARTESIAN_POINT('Ctrl Pts',(-18.7782261525852,-21.5130968722283,
-2.36886253713868));
#64800=CARTESIAN_POINT('Ctrl Pts',(-18.8652810139474,-21.5101090568401,
-2.37317869984855));
#64801=CARTESIAN_POINT('Ctrl Pts',(-18.9518945613347,-21.5027100893949,
-2.37749486255842));
#64802=CARTESIAN_POINT('Ctrl Pts',(-19.0356866828293,-21.4955521424246,
-2.38167042678695));
#64803=CARTESIAN_POINT('Ctrl Pts',(-19.1190653399573,-21.4842661264592,
-2.38584599101548));
#64804=CARTESIAN_POINT('Ctrl Pts',(-19.2015998086145,-21.4689327402582,
-2.39002155524401));
#64805=CARTESIAN_POINT('Ctrl Pts',(-19.2883028950859,-21.4528249015417,
-2.39440801719455));
#64806=CARTESIAN_POINT('Ctrl Pts',(-19.3740737042372,-21.4322502184736,
-2.39879447914509));
#64807=CARTESIAN_POINT('Ctrl Pts',(-19.4584303876454,-21.4073616054374,
-2.40318094109563));
#64808=CARTESIAN_POINT('Ctrl Pts',(-19.5427870710536,-21.3824729924011,
-2.40756740304617));
#64809=CARTESIAN_POINT('Ctrl Pts',(-19.6257291066931,-21.3532707138335,
-2.41195386499671));
#64810=CARTESIAN_POINT('Ctrl Pts',(-19.7068005673137,-21.3199651720906,
-2.41634032694725));
#64811=CARTESIAN_POINT('Ctrl Pts',(-19.7841418063303,-21.2881920691418,
-2.42052496109048));
#64812=CARTESIAN_POINT('Ctrl Pts',(-19.8600687027268,-21.2525667345391,
-2.4247095952337));
#64813=CARTESIAN_POINT('Ctrl Pts',(-19.9341709431478,-21.2132363227278,
-2.42889422937693));
#64814=CARTESIAN_POINT('Ctrl Pts',(-20.0081677081176,-21.1739618929342,
-2.43307290720666));
#64815=CARTESIAN_POINT('Ctrl Pts',(-20.0803445730473,-21.1309930750319,
-2.4372515850364));
#64816=CARTESIAN_POINT('Ctrl Pts',(-20.1503107695072,-21.0845252177121,
-2.44143026286614));
#64817=CARTESIAN_POINT('Ctrl Pts',(-20.2215310651425,-21.0372244538674,
-2.44568384081458));
#64818=CARTESIAN_POINT('Ctrl Pts',(-20.2904602140006,-20.9862981588784,
-2.44993741876302));
#64819=CARTESIAN_POINT('Ctrl Pts',(-20.3567118459237,-20.932001582095,-2.45419099671146));
#64820=CARTESIAN_POINT('Ctrl Pts',(-20.4216790556215,-20.8787576545515,
-2.45836211042625));
#64821=CARTESIAN_POINT('Ctrl Pts',(-20.4840712679219,-20.8222732635721,
-2.46253322414104));
#64822=CARTESIAN_POINT('Ctrl Pts',(-20.5435545161742,-20.7628319781232,
-2.46670433785583));
#64823=CARTESIAN_POINT('Ctrl Pts',(-20.6030178042074,-20.7034106388123,
-2.47087405191028));
#64824=CARTESIAN_POINT('Ctrl Pts',(-20.6595737416717,-20.6410347004966,
-2.47504376596472));
#64825=CARTESIAN_POINT('Ctrl Pts',(-20.7129241773316,-20.5760255848885,
-2.47921348001916));
#64826=CARTESIAN_POINT('Ctrl Pts',(-20.7662727145228,-20.5110187826217,
-2.48338304569485));
#64827=CARTESIAN_POINT('Ctrl Pts',(-20.8164156855257,-20.4433793455188,
-2.48755261137053));
#64828=CARTESIAN_POINT('Ctrl Pts',(-20.8630951945853,-20.3734618012432,
-2.49172217704622));
#64829=CARTESIAN_POINT('Ctrl Pts',(-20.9114159041743,-20.3010860325135,
-2.49603834009476));
#64830=CARTESIAN_POINT('Ctrl Pts',(-20.9560247758173,-20.226269417489,-2.5003545031433));
#64831=CARTESIAN_POINT('Ctrl Pts',(-20.9966856911225,-20.1494362042253,
-2.50467066619184));
#64832=CARTESIAN_POINT('Ctrl Pts',(-21.036022076007,-20.0751058349709,-2.50884623011182));
#64833=CARTESIAN_POINT('Ctrl Pts',(-21.0716636082435,-19.9988886784647,
-2.5130217940318));
#64834=CARTESIAN_POINT('Ctrl Pts',(-21.1034449999269,-19.9211905861704,
-2.51719735795179));
#64835=CARTESIAN_POINT('Ctrl Pts',(-21.1368316008925,-19.839568131463,-2.52158382056461));
#64836=CARTESIAN_POINT('Ctrl Pts',(-21.1659576672678,-19.756311755636,-2.52597028317742));
#64837=CARTESIAN_POINT('Ctrl Pts',(-21.1906909603509,-19.6719093868885,
-2.53035674579024));
#64838=CARTESIAN_POINT('Ctrl Pts',(-21.215424253434,-19.5875070181411,-2.53474320840306));
#64839=CARTESIAN_POINT('Ctrl Pts',(-21.2357647130118,-19.5019592385496,
-2.53912967101588));
#64840=CARTESIAN_POINT('Ctrl Pts',(-21.2516424693651,-19.4157632978678,
-2.54351613362869));
#64841=CARTESIAN_POINT('Ctrl Pts',(-21.2744558895146,-19.2919155598001,
-2.54981867489014));
#64842=CARTESIAN_POINT('Ctrl Pts',(-21.2881358177162,-19.1663368452798,
-2.55612121615159));
#64843=CARTESIAN_POINT('Ctrl Pts',(-21.2924829866165,-19.0401181433864,
-2.56242375741304));
#64844=CARTESIAN_POINT('Ctrl Pts',(-21.2934684379609,-19.0115058689788,
-2.56385246835153));
#64845=CARTESIAN_POINT('Ctrl Pts',(-21.2939744691011,-18.982860830915,-2.56528117929002));
#64846=CARTESIAN_POINT('Ctrl Pts',(-21.2939990581247,-18.9541959965425,
-2.56670989022851));
#64847=CARTESIAN_POINT('Origin',(-18.734,-18.952,1.76670989022851));
#64848=CARTESIAN_POINT('',(-17.1744641548914,-16.9218650419685,-1.2500388607805));
#64849=CARTESIAN_POINT('',(-17.1763037562513,-16.9242236971174,-1.31677679576761));
#64850=CARTESIAN_POINT('',(-17.1744641548914,-16.9218650419685,1.76670989022851));
#64851=CARTESIAN_POINT('',(-21.2937660511389,-18.9530076677181,-1.83329006740113));
#64852=CARTESIAN_POINT('Ctrl Pts',(-17.1763037562512,-16.9242236971175,
-1.31677679576762));
#64853=CARTESIAN_POINT('Ctrl Pts',(-16.7482596907349,-17.2576787930677,
-1.34369096971429));
#64854=CARTESIAN_POINT('Ctrl Pts',(-15.9020682097871,-18.4571854904752,
-1.41299707922144));
#64855=CARTESIAN_POINT('Ctrl Pts',(-16.4540143580209,-20.9432205748173,
-1.52469512428907));
#64856=CARTESIAN_POINT('Ctrl Pts',(-19.1741877112253,-21.9469162432243,
-1.65187093097051));
#64857=CARTESIAN_POINT('Ctrl Pts',(-21.0477247446925,-20.5363391578402,
-1.75473569408639));
#64858=CARTESIAN_POINT('Ctrl Pts',(-21.2914430930582,-19.3178333754147,
-1.81520852164178));
#64859=CARTESIAN_POINT('Ctrl Pts',(-21.2901593318677,-18.9530194399495,
-1.8332894136367));
#64860=CARTESIAN_POINT('Ctrl Pts',(-21.293999801981,-18.9530069047618,-1.83329010977149));
#64861=CARTESIAN_POINT('Ctrl Pts',(-21.2940336318731,-18.8669962707737,
-1.83754657623943));
#64862=CARTESIAN_POINT('Ctrl Pts',(-21.2897284501564,-18.7810104793984,
-1.84180304270736));
#64863=CARTESIAN_POINT('Ctrl Pts',(-21.2811180404876,-18.6955049945465,
-1.8460595091753));
#64864=CARTESIAN_POINT('Ctrl Pts',(-21.272502628509,-18.6099498343665,-1.85031844848306));
#64865=CARTESIAN_POINT('Ctrl Pts',(-21.2595770560965,-18.5248759662227,
-1.85457738779083));
#64866=CARTESIAN_POINT('Ctrl Pts',(-21.2424267247842,-18.4407316102198,
-1.8588363270986));
#64867=CARTESIAN_POINT('Ctrl Pts',(-21.2252479656664,-18.3564477793963,
-1.8631023258792));
#64868=CARTESIAN_POINT('Ctrl Pts',(-21.2038305496871,-18.273096962458,-1.8673683246598));
#64869=CARTESIAN_POINT('Ctrl Pts',(-21.1783105998859,-18.191115191842,-1.87163432344041));
#64870=CARTESIAN_POINT('Ctrl Pts',(-21.1527682035212,-18.1090613125802,
-1.87590407446243));
#64871=CARTESIAN_POINT('Ctrl Pts',(-21.1231162337396,-18.0283792845701,
-1.88017382548446));
#64872=CARTESIAN_POINT('Ctrl Pts',(-21.0895392521437,-17.949485744934,-1.88444357650648));
#64873=CARTESIAN_POINT('Ctrl Pts',(-21.0558918636089,-17.8704267749242,
-1.88872228068881));
#64874=CARTESIAN_POINT('Ctrl Pts',(-21.0183032087881,-17.7931641756621,
-1.89300098487114));
#64875=CARTESIAN_POINT('Ctrl Pts',(-20.9770042486984,-17.7180907892714,
-1.89727968905346));
#64876=CARTESIAN_POINT('Ctrl Pts',(-20.9482314701846,-17.6657875372232,
-1.90026064081344));
#64877=CARTESIAN_POINT('Ctrl Pts',(-20.917658721245,-17.614546342522,-1.90324159257341));
#64878=CARTESIAN_POINT('Ctrl Pts',(-20.8853760799725,-17.5644910946152,
-1.90622254433338));
#64879=CARTESIAN_POINT('Ctrl Pts',(-20.8400579766697,-17.4942239539453,
-1.91040717961954));
#64880=CARTESIAN_POINT('Ctrl Pts',(-20.7912093745918,-17.4260486192458,
-1.9145918149057));
#64881=CARTESIAN_POINT('Ctrl Pts',(-20.7390496453448,-17.3603417704474,
-1.91877645019186));
#64882=CARTESIAN_POINT('Ctrl Pts',(-20.6869641588708,-17.294728447032,-1.92295512917932));
#64883=CARTESIAN_POINT('Ctrl Pts',(-20.6315771902452,-17.2315769876738,
-1.92713380816678));
#64884=CARTESIAN_POINT('Ctrl Pts',(-20.5731519433967,-17.1712360827161,
-1.93131248715424));
#64885=CARTESIAN_POINT('Ctrl Pts',(-20.513679481987,-17.1098136269271,-1.9355660648151));
#64886=CARTESIAN_POINT('Ctrl Pts',(-20.4510590117389,-17.05130387858,-1.93981964247596));
#64887=CARTESIAN_POINT('Ctrl Pts',(-20.3856118360818,-16.9960403013062,
-1.94407322013681));
#64888=CARTESIAN_POINT('Ctrl Pts',(-20.321433464053,-16.94184810147,-1.94824433503721));
#64889=CARTESIAN_POINT('Ctrl Pts',(-20.2545373771257,-16.8907776413735,
-1.9524154499376));
#64890=CARTESIAN_POINT('Ctrl Pts',(-20.1852631886002,-16.8431057026456,
-1.95658656483799));
#64891=CARTESIAN_POINT('Ctrl Pts',(-20.1160122456088,-16.7954497606359,
-1.96075628008585));
#64892=CARTESIAN_POINT('Ctrl Pts',(-20.0443851644975,-16.751190335713,-1.96492599533372));
#64893=CARTESIAN_POINT('Ctrl Pts',(-19.9707522609747,-16.7105621032529,
-1.96909571058158));
#64894=CARTESIAN_POINT('Ctrl Pts',(-19.8971219775585,-16.6699353164821,
-1.97326527745694));
#64895=CARTESIAN_POINT('Ctrl Pts',(-19.8214864168391,-16.6329396867698,
-1.9774348443323));
#64896=CARTESIAN_POINT('Ctrl Pts',(-19.7442411213498,-16.5997642812138,
-1.98160441120766));
#64897=CARTESIAN_POINT('Ctrl Pts',(-19.6642800145859,-16.5654224856546,
-1.98592057285825));
#64898=CARTESIAN_POINT('Ctrl Pts',(-19.5825943566344,-16.5351747549186,
-1.99023673450885));
#64899=CARTESIAN_POINT('Ctrl Pts',(-19.4996442818956,-16.5091760534986,
-1.99455289615945));
#64900=CARTESIAN_POINT('Ctrl Pts',(-19.4193962589829,-16.4840242450908,
-1.99872846128247));
#64901=CARTESIAN_POINT('Ctrl Pts',(-19.3379653976298,-16.462848969509,-2.0029040264055));
#64902=CARTESIAN_POINT('Ctrl Pts',(-19.2557808529988,-16.4457388920059,
-2.00707959152852));
#64903=CARTESIAN_POINT('Ctrl Pts',(-19.169445422947,-16.4277646377701,-2.01146605144291));
#64904=CARTESIAN_POINT('Ctrl Pts',(-19.082278749795,-16.414277123413,-2.01585251135729));
#64905=CARTESIAN_POINT('Ctrl Pts',(-18.9947846786654,-16.4053175794039,
-2.02023897127167));
#64906=CARTESIAN_POINT('Ctrl Pts',(-18.9072906075359,-16.3963580353947,
-2.02462543118606));
#64907=CARTESIAN_POINT('Ctrl Pts',(-18.8194697217397,-16.3919264150073,
-2.02901189110044));
#64908=CARTESIAN_POINT('Ctrl Pts',(-18.7318236815548,-16.3920009250709,
-2.03339835101482));
#64909=CARTESIAN_POINT('Ctrl Pts',(-18.6482254298241,-16.3920719940095,
-2.03758222948047));
#64910=CARTESIAN_POINT('Ctrl Pts',(-18.5644751184203,-16.3962424237152,
-2.04176610794612));
#64911=CARTESIAN_POINT('Ctrl Pts',(-18.481007980681,-16.4045316413818,-2.04594998641176));
#64912=CARTESIAN_POINT('Ctrl Pts',(-18.3976520608444,-16.4128098138703,
-2.05012828996254));
#64913=CARTESIAN_POINT('Ctrl Pts',(-18.3145790190413,-16.4251958328771,
-2.05430659351331));
#64914=CARTESIAN_POINT('Ctrl Pts',(-18.2322243990186,-16.4416571456752,
-2.05848489706408));
#64915=CARTESIAN_POINT('Ctrl Pts',(-18.1499547982016,-16.4581014645543,
-2.06265888712218));
#64916=CARTESIAN_POINT('Ctrl Pts',(-18.0684025947205,-16.478612631518,-2.06683287718028));
#64917=CARTESIAN_POINT('Ctrl Pts',(-17.987997155221,-16.5031064221609,-2.07100686723839));
#64918=CARTESIAN_POINT('Ctrl Pts',(-17.9076457851775,-16.527583741705,-2.0751780504544));
#64919=CARTESIAN_POINT('Ctrl Pts',(-17.8284400864782,-16.5560382324587,
-2.07934923367041));
#64920=CARTESIAN_POINT('Ctrl Pts',(-17.7507969267065,-16.5883351090592,
-2.08352041688642));
#64921=CARTESIAN_POINT('Ctrl Pts',(-17.6731854101898,-16.620618823157,-2.08768990014826));
#64922=CARTESIAN_POINT('Ctrl Pts',(-17.5971355906324,-16.6567416327186,
-2.09185938341009));
#64923=CARTESIAN_POINT('Ctrl Pts',(-17.5230455881934,-16.6965201369717,
-2.09602886667192));
#64924=CARTESIAN_POINT('Ctrl Pts',(-17.448941785493,-16.7363060505073,-2.10019912655621));
#64925=CARTESIAN_POINT('Ctrl Pts',(-17.3767989370841,-16.7797488058129,
-2.10436938644049));
#64926=CARTESIAN_POINT('Ctrl Pts',(-17.3069908375485,-16.8266188929325,
-2.10853964632478));
#64927=CARTESIAN_POINT('Ctrl Pts',(-17.2618060573289,-16.8569565557462,
-2.11123893591414));
#64928=CARTESIAN_POINT('Ctrl Pts',(-17.217598927097,-16.8887292038021,-2.11393822550351));
#64929=CARTESIAN_POINT('Ctrl Pts',(-17.1744641548914,-16.9218650419685,
-2.11663751509287));
#64930=CARTESIAN_POINT('',(-21.2939995273704,-18.9504444089713,-1.76670989019937));
#64931=CARTESIAN_POINT('Ctrl Pts',(-21.29399952737,-18.9504444083884,-1.7667098902285));
#64932=CARTESIAN_POINT('Ctrl Pts',(-21.2939437779003,-18.8586988530854,
-1.77129369133236));
#64933=CARTESIAN_POINT('Ctrl Pts',(-21.2889563823031,-18.7671041917188,
-1.77587749243622));
#64934=CARTESIAN_POINT('Ctrl Pts',(-21.2790836671927,-18.6760486872856,
-1.78046129354008));
#64935=CARTESIAN_POINT('Ctrl Pts',(-21.2700706759119,-18.5929223680962,
-1.78464593362342));
#64936=CARTESIAN_POINT('Ctrl Pts',(-21.2569640808322,-18.5100833893621,
-1.78883057370677));
#64937=CARTESIAN_POINT('Ctrl Pts',(-21.2397911341478,-18.4279668025532,
-1.79301521379011));
#64938=CARTESIAN_POINT('Ctrl Pts',(-21.2226426307479,-18.3459670972049,
-1.79719389762437));
#64939=CARTESIAN_POINT('Ctrl Pts',(-21.2014393656626,-18.2646881878446,
-1.80137258145863));
#64940=CARTESIAN_POINT('Ctrl Pts',(-21.1762603194833,-18.1845597535461,
-1.80555126529289));
#64941=CARTESIAN_POINT('Ctrl Pts',(-21.1506300008844,-18.1029952143143,
-1.80980484174825));
#64942=CARTESIAN_POINT('Ctrl Pts',(-21.1208800336003,-18.0226232755941,
-1.81405841820361));
#64943=CARTESIAN_POINT('Ctrl Pts',(-21.0871481586077,-17.9438860463016,
-1.81831199465897));
#64944=CARTESIAN_POINT('Ctrl Pts',(-21.0540701842775,-17.866675157493,-1.82248311449243));
#64945=CARTESIAN_POINT('Ctrl Pts',(-21.0171634947162,-17.7910366074843,
-1.82665423432589));
#64946=CARTESIAN_POINT('Ctrl Pts',(-20.9766076064455,-17.7173700459194,
-1.83082535415935));
#64947=CARTESIAN_POINT('Ctrl Pts',(-20.9360653268187,-17.6437282033794,
-1.83499507436165));
#64948=CARTESIAN_POINT('Ctrl Pts',(-20.8918765020354,-17.5720574377846,
-1.83916479456395));
#64949=CARTESIAN_POINT('Ctrl Pts',(-20.8442669678557,-17.5027335219578,
-1.84333451476625));
#64950=CARTESIAN_POINT('Ctrl Pts',(-20.7966591276122,-17.4334120726597,
-1.84750408661088));
#64951=CARTESIAN_POINT('Ctrl Pts',(-20.7456310810944,-17.3664376858416,
-1.8516736584555));
#64952=CARTESIAN_POINT('Ctrl Pts',(-20.6914516584179,-17.3021566726028,
-1.85584323030013));
#64953=CARTESIAN_POINT('Ctrl Pts',(-20.6353675232618,-17.2356158189659,
-1.86015938612691));
#64954=CARTESIAN_POINT('Ctrl Pts',(-20.5759066443104,-17.1719616467127,
-1.8644755419537));
#64955=CARTESIAN_POINT('Ctrl Pts',(-20.5134108747745,-17.111538933111,-1.86879169778048));
#64956=CARTESIAN_POINT('Ctrl Pts',(-20.4529507162969,-17.0530843070278,
-1.87296726785888));
#64957=CARTESIAN_POINT('Ctrl Pts',(-20.3896507223166,-16.9976541361553,
-1.87714283793729));
#64958=CARTESIAN_POINT('Ctrl Pts',(-20.3238547745764,-16.9455200485037,
-1.88131840801569));
#64959=CARTESIAN_POINT('Ctrl Pts',(-20.2547359371302,-16.8907530354344,
-1.88570485671667));
#64960=CARTESIAN_POINT('Ctrl Pts',(-20.182862878563,-16.8396241326094,-1.89009130541764));
#64961=CARTESIAN_POINT('Ctrl Pts',(-20.1086675044515,-16.7923960427418,
-1.89447775411861));
#64962=CARTESIAN_POINT('Ctrl Pts',(-20.03447213034,-16.7451679528743,-1.89886420281958));
#64963=CARTESIAN_POINT('Ctrl Pts',(-19.9579549830438,-16.7018408956605,
-1.90325065152055));
#64964=CARTESIAN_POINT('Ctrl Pts',(-19.8795742651273,-16.6626202580004,
-1.90763710022152));
#64965=CARTESIAN_POINT('Ctrl Pts',(-19.8047997208725,-16.6252041002467,
-1.91182173531074));
#64966=CARTESIAN_POINT('Ctrl Pts',(-19.7280509965214,-16.5913855369158,
-1.91600637039996));
#64967=CARTESIAN_POINT('Ctrl Pts',(-19.649708651428,-16.5613771385474,-1.92019100548918));
#64968=CARTESIAN_POINT('Ctrl Pts',(-19.5714778164139,-16.5314114532082,
-1.92436968429779));
#64969=CARTESIAN_POINT('Ctrl Pts',(-19.4916582921575,-16.5052453236535,
-1.9285483631064));
#64970=CARTESIAN_POINT('Ctrl Pts',(-19.4106541203679,-16.4830449170977,
-1.93272704191501));
#64971=CARTESIAN_POINT('Ctrl Pts',(-19.3281980247581,-16.4604465890721,
-1.93698061962285));
#64972=CARTESIAN_POINT('Ctrl Pts',(-19.2445148259725,-16.4419577675855,
-1.94123419733068));
#64973=CARTESIAN_POINT('Ctrl Pts',(-19.1600508251799,-16.4277019402686,
-1.94548777503851));
#64974=CARTESIAN_POINT('Ctrl Pts',(-19.0772243047194,-16.4137224867517,
-1.94965888980624));
#64975=CARTESIAN_POINT('Ctrl Pts',(-18.9936474609865,-16.4038134443357,
-1.95383000457398));
#64976=CARTESIAN_POINT('Ctrl Pts',(-18.9097535040447,-16.3980401910335,
-1.95800111934171));
#64977=CARTESIAN_POINT('Ctrl Pts',(-18.8258876980693,-16.3922688749706,
-1.96217083447453));
#64978=CARTESIAN_POINT('Ctrl Pts',(-18.7417054487798,-16.3906306234225,
-1.96634054960734));
#64979=CARTESIAN_POINT('Ctrl Pts',(-18.6576449613786,-16.3931389431864,
-1.97051026474016));
#64980=CARTESIAN_POINT('Ctrl Pts',(-18.5735874647729,-16.3956471737067,
-1.97467983151832));
#64981=CARTESIAN_POINT('Ctrl Pts',(-18.4896521812446,-16.4023016676361,
-1.97884939829647));
#64982=CARTESIAN_POINT('Ctrl Pts',(-18.4062758154027,-16.4130638332502,
-1.98301896507463));
#64983=CARTESIAN_POINT('Ctrl Pts',(-18.319968075054,-16.4242043787278,-1.98733512689366));
#64984=CARTESIAN_POINT('Ctrl Pts',(-18.2342598093425,-16.439746750557,-1.99165128871268));
#64985=CARTESIAN_POINT('Ctrl Pts',(-18.1496259627856,-16.4595901250738,
-1.99596745053171));
#64986=CARTESIAN_POINT('Ctrl Pts',(-18.0677490201717,-16.4787871118902,
-2.00014301560344));
#64987=CARTESIAN_POINT('Ctrl Pts',(-17.9868780138239,-16.502009022233,-2.00431858067517));
#64988=CARTESIAN_POINT('Ctrl Pts',(-17.9074274756713,-16.5291137331635,
-2.0084941457469));
#64989=CARTESIAN_POINT('Ctrl Pts',(-17.8239641319307,-16.5575874207934,
-2.01288060593957));
#64990=CARTESIAN_POINT('Ctrl Pts',(-17.742069063372,-16.590346235575,-2.01726706613225));
#64991=CARTESIAN_POINT('Ctrl Pts',(-17.662196947742,-16.6271692067657,-2.02165352632493));
#64992=CARTESIAN_POINT('Ctrl Pts',(-17.5823248321119,-16.6639921779564,
-2.0260399865176));
#64993=CARTESIAN_POINT('Ctrl Pts',(-17.504476147719,-16.7048789684268,-2.03042644671028));
#64994=CARTESIAN_POINT('Ctrl Pts',(-17.4290716122241,-16.7495554711238,
-2.03481290690295));
#64995=CARTESIAN_POINT('Ctrl Pts',(-17.3571349233601,-16.792177306176,-2.03899763425421));
#64996=CARTESIAN_POINT('Ctrl Pts',(-17.2871547394863,-16.8384065836607,
-2.04318236160547));
#64997=CARTESIAN_POINT('Ctrl Pts',(-17.2195158141186,-16.8880383601638,
-2.04736708895673));
#64998=CARTESIAN_POINT('Ctrl Pts',(-17.2043800615047,-16.8991446024179,
-2.04830351716876));
#64999=CARTESIAN_POINT('Ctrl Pts',(-17.1893614580268,-16.9104210351831,
-2.04923994538079));
#65000=CARTESIAN_POINT('Ctrl Pts',(-17.1744641548914,-16.9218650419685,
-2.05017637359282));
#65001=CARTESIAN_POINT('Ctrl Pts',(-17.1744641548914,-16.9218650419685,
-1.2500388607805));
#65002=CARTESIAN_POINT('Ctrl Pts',(-17.1078165570043,-16.9730632726498,
-1.25422272801441));
#65003=CARTESIAN_POINT('Ctrl Pts',(-17.0437742835163,-17.0274842711545,
-1.25840659524833));
#65004=CARTESIAN_POINT('Ctrl Pts',(-16.9826475255332,-17.0848191008424,
-1.26259046248224));
#65005=CARTESIAN_POINT('Ctrl Pts',(-16.9380009581382,-17.1266960696561,
-1.26564633059294));
#65006=CARTESIAN_POINT('Ctrl Pts',(-16.8949089970119,-17.1701266834957,
-1.26870219870364));
#65007=CARTESIAN_POINT('Ctrl Pts',(-16.8534788456906,-17.2149795084125,
-1.27175806681434));
#65008=CARTESIAN_POINT('Ctrl Pts',(-16.7967468035303,-17.2763983609397,
-1.2759425950616));
#65009=CARTESIAN_POINT('Ctrl Pts',(-16.7429212561054,-17.3407138418484,
-1.28012712330885));
#65010=CARTESIAN_POINT('Ctrl Pts',(-16.6923122163234,-17.4076195436403,
-1.28431165155611));
#65011=CARTESIAN_POINT('Ctrl Pts',(-16.6417752336977,-17.4744299850868,
-1.2884902218716));
#65012=CARTESIAN_POINT('Ctrl Pts',(-16.5944459372434,-17.5438229582135,
-1.29266879218709));
#65013=CARTESIAN_POINT('Ctrl Pts',(-16.5505962988509,-17.6154565933691,
-1.29684736250257));
#65014=CARTESIAN_POINT('Ctrl Pts',(-16.5059592554184,-17.6883765489466,
-1.30110096712729));
#65015=CARTESIAN_POINT('Ctrl Pts',(-16.4649284015663,-17.7636180793202,
-1.30535457175201));
#65016=CARTESIAN_POINT('Ctrl Pts',(-16.4277464893493,-17.8407868140581,
-1.30960817637672));
#65017=CARTESIAN_POINT('Ctrl Pts',(-16.3912866203068,-17.9164569933188,
-1.31377917938137));
#65018=CARTESIAN_POINT('Ctrl Pts',(-16.3585277513987,-17.9939797629346,
-1.31795018238602));
#65019=CARTESIAN_POINT('Ctrl Pts',(-16.3296531528721,-18.0729572031431,
-1.32212118539066));
#65020=CARTESIAN_POINT('Ctrl Pts',(-16.3007882503651,-18.1519081229202,
-1.32629078778269));
#65021=CARTESIAN_POINT('Ctrl Pts',(-16.2758051856693,-18.2323123114455,
-1.33046039017473));
#65022=CARTESIAN_POINT('Ctrl Pts',(-16.2548387934267,-18.3137526249001,
-1.33462999256676));
#65023=CARTESIAN_POINT('Ctrl Pts',(-16.2338731513477,-18.3951900244743,
-1.33879944577318));
#65024=CARTESIAN_POINT('Ctrl Pts',(-16.2169240098583,-18.477663029525,-1.3429688989796));
#65025=CARTESIAN_POINT('Ctrl Pts',(-16.2040757430117,-18.5607414487807,
-1.34713835218602));
#65026=CARTESIAN_POINT('Ctrl Pts',(-16.1907749845688,-18.6467457324343,
-1.3514546456285));
#65027=CARTESIAN_POINT('Ctrl Pts',(-16.181869424783,-18.7333983482173,-1.35577093907098));
#65028=CARTESIAN_POINT('Ctrl Pts',(-16.1773942991259,-18.8202149846984,
-1.36008723251346));
#65029=CARTESIAN_POINT('Ctrl Pts',(-16.1730651991088,-18.90419874991,-1.36426268309241));
#65030=CARTESIAN_POINT('Ctrl Pts',(-16.1728817996142,-18.9883355251162,
-1.36843813367136));
#65031=CARTESIAN_POINT('Ctrl Pts',(-16.1768228581885,-19.0721876258056,
-1.37261358425031));
#65032=CARTESIAN_POINT('Ctrl Pts',(-16.1809633215807,-19.1602823716003,
-1.37700029912456));
#65033=CARTESIAN_POINT('Ctrl Pts',(-16.1896565615449,-19.2480622945844,
-1.3813870139988));
#65034=CARTESIAN_POINT('Ctrl Pts',(-16.2028167371298,-19.3350290978058,
-1.38577372887305));
#65035=CARTESIAN_POINT('Ctrl Pts',(-16.2159769127148,-19.4219959010273,
-1.39016044374729));
#65036=CARTESIAN_POINT('Ctrl Pts',(-16.2336038329925,-19.5081490310293,
-1.39454715862153));
#65037=CARTESIAN_POINT('Ctrl Pts',(-16.2555511525982,-19.593008042705,-1.39893387349578));
#65038=CARTESIAN_POINT('Ctrl Pts',(-16.276487610888,-19.6739585729016,-1.40311854272393));
#65039=CARTESIAN_POINT('Ctrl Pts',(-16.3014331778146,-19.7540329167562,
-1.40730321195209));
#65040=CARTESIAN_POINT('Ctrl Pts',(-16.3302979840591,-19.8328045291445,
-1.41148788118024));
#65041=CARTESIAN_POINT('Ctrl Pts',(-16.3591217073558,-19.9114640268001,
-1.41566659441667));
#65042=CARTESIAN_POINT('Ctrl Pts',(-16.3918534329631,-19.988824047698,-1.4198453076531));
#65043=CARTESIAN_POINT('Ctrl Pts',(-16.4283528834957,-20.064470841935,-1.42402402088953));
#65044=CARTESIAN_POINT('Ctrl Pts',(-16.4655061714862,-20.1414727444521,
-1.42827759002651));
#65045=CARTESIAN_POINT('Ctrl Pts',(-16.506563383349,-20.2166989674673,-1.4325311591635));
#65046=CARTESIAN_POINT('Ctrl Pts',(-16.551324307012,-20.2897319683851,-1.43678472830049));
#65047=CARTESIAN_POINT('Ctrl Pts',(-16.595217918491,-20.3613498418582,-1.4409558779511));
#65048=CARTESIAN_POINT('Ctrl Pts',(-16.642672740131,-20.430858319068,-1.44512702760171));
#65049=CARTESIAN_POINT('Ctrl Pts',(-16.6934533571751,-20.4978878997056,
-1.44929817725232));
#65050=CARTESIAN_POINT('Ctrl Pts',(-16.7442169358474,-20.564894989972,-1.45346792736108));
#65051=CARTESIAN_POINT('Ctrl Pts',(-16.7983038161653,-20.6294244691448,
-1.45763767746983));
#65052=CARTESIAN_POINT('Ctrl Pts',(-16.8554362029378,-20.6911371597339,
-1.46180742757859));
#65053=CARTESIAN_POINT('Ctrl Pts',(-16.9125665576473,-20.7528476553495,
-1.46597702937926));
#65054=CARTESIAN_POINT('Ctrl Pts',(-16.9727418902975,-20.8117412245847,
-1.47014663117994));
#65055=CARTESIAN_POINT('Ctrl Pts',(-17.0356461226138,-20.8675140582014,
-1.47431623298061));
#65056=CARTESIAN_POINT('Ctrl Pts',(-17.100760794443,-20.9252467357051,-1.47863235358033));
#65057=CARTESIAN_POINT('Ctrl Pts',(-17.1687993304482,-20.9796349174704,
-1.48294847418005));
#65058=CARTESIAN_POINT('Ctrl Pts',(-17.2393736359262,-21.0303868821313,
-1.48726459477976));
#65059=CARTESIAN_POINT('Ctrl Pts',(-17.3076502404839,-21.0794865055453,
-1.49144019463036));
#65060=CARTESIAN_POINT('Ctrl Pts',(-17.3782996119825,-21.1251828324923,
-1.49561579448095));
#65061=CARTESIAN_POINT('Ctrl Pts',(-17.4509422068433,-21.1672568021383,
-1.49979139433154));
#65062=CARTESIAN_POINT('Ctrl Pts',(-17.5272517449746,-21.2114546339639,
-1.50417777530582));
#65063=CARTESIAN_POINT('Ctrl Pts',(-17.6057605149863,-21.2516545112966,
-1.5085641562801));
#65064=CARTESIAN_POINT('Ctrl Pts',(-17.6860031954809,-21.2876589429362,
-1.51295053725438));
#65065=CARTESIAN_POINT('Ctrl Pts',(-17.7662458759755,-21.3236633745758,
-1.51733691822866));
#65066=CARTESIAN_POINT('Ctrl Pts',(-17.8482218986034,-21.3554722215575,
-1.52172329920294));
#65067=CARTESIAN_POINT('Ctrl Pts',(-17.9314482087024,-21.3829485025983,
-1.52610968017722));
#65068=CARTESIAN_POINT('Ctrl Pts',(-18.01084679095,-21.4091611000027,-1.53029432359276));
#65069=CARTESIAN_POINT('Ctrl Pts',(-18.0916786888191,-21.4315284615327,
-1.53447896700831));
#65070=CARTESIAN_POINT('Ctrl Pts',(-18.1735366063454,-21.4498952708977,
-1.53866361042385));
#65071=CARTESIAN_POINT('Ctrl Pts',(-18.2552780145749,-21.4682359385759,
-1.54284229778925));
#65072=CARTESIAN_POINT('Ctrl Pts',(-18.3380420967243,-21.4825872643746,
-1.54702098515466));
#65073=CARTESIAN_POINT('Ctrl Pts',(-18.4214050302511,-21.4928432428797,
-1.55119967252006));
#65074=CARTESIAN_POINT('Ctrl Pts',(-18.5062619503251,-21.5032830236249,
-1.5554532481175));
#65075=CARTESIAN_POINT('Ctrl Pts',(-18.5917389405056,-21.5094790670787,
-1.55970682371494));
#65076=CARTESIAN_POINT('Ctrl Pts',(-18.6773765369535,-21.5113737092173,
-1.56396039931238));
#65077=CARTESIAN_POINT('Ctrl Pts',(-18.7613541250249,-21.513231625409,-1.56813152314313));
#65078=CARTESIAN_POINT('Ctrl Pts',(-18.8454856674055,-21.510953399411,-1.57230264697389));
#65079=CARTESIAN_POINT('Ctrl Pts',(-18.9293330517837,-21.5045369730683,
-1.57647377080464));
#65080=CARTESIAN_POINT('Ctrl Pts',(-19.0131523042948,-21.4981226995185,
-1.58064349517013));
#65081=CARTESIAN_POINT('Ctrl Pts',(-19.0966871298398,-21.4875730181186,
-1.58481321953563));
#65082=CARTESIAN_POINT('Ctrl Pts',(-19.179501972955,-21.4729379191272,-1.58898294390113));
#65083=CARTESIAN_POINT('Ctrl Pts',(-19.2623138727389,-21.4583033402833,
-1.59315252007));
#65084=CARTESIAN_POINT('Ctrl Pts',(-19.3444053881076,-21.4395837134394,
-1.59732209623888));
#65085=CARTESIAN_POINT('Ctrl Pts',(-19.4253499807632,-21.4168803630397,
-1.60149167240775));
#65086=CARTESIAN_POINT('Ctrl Pts',(-19.5091400560411,-21.3933789112856,
-1.60580782361199));
#65087=CARTESIAN_POINT('Ctrl Pts',(-19.5917005611986,-21.3656085745896,
-1.61012397481624));
#65088=CARTESIAN_POINT('Ctrl Pts',(-19.6725761234496,-21.3337377816398,
-1.61444012602048));
#65089=CARTESIAN_POINT('Ctrl Pts',(-19.7508175799528,-21.3029050159575,
-1.61861570078383));
#65090=CARTESIAN_POINT('Ctrl Pts',(-19.8274817556368,-21.2682350333859,
-1.62279127554719));
#65091=CARTESIAN_POINT('Ctrl Pts',(-19.9021790201189,-21.2299283959234,
-1.62696685031055));
#65092=CARTESIAN_POINT('Ctrl Pts',(-19.9806484631081,-21.1896872903713,
-1.63135328973523));
#65093=CARTESIAN_POINT('Ctrl Pts',(-20.0569466040008,-21.1454328549357,
-1.63573972915991));
#65094=CARTESIAN_POINT('Ctrl Pts',(-20.1306554964563,-21.0974494690434,
-1.6401261685846));
#65095=CARTESIAN_POINT('Ctrl Pts',(-20.2043643889117,-21.049466083151,-1.64451260800928));
#65096=CARTESIAN_POINT('Ctrl Pts',(-20.2754836084046,-20.9977541495255,
-1.64889904743396));
#65097=CARTESIAN_POINT('Ctrl Pts',(-20.34363649293,-20.9426457144927,-1.65328548685865));
#65098=CARTESIAN_POINT('Ctrl Pts',(-20.4078056269716,-20.8907585408379,
-1.65741552510087));
#65099=CARTESIAN_POINT('Ctrl Pts',(-20.469597781961,-20.8356563927705,-1.6615455633431));
#65100=CARTESIAN_POINT('Ctrl Pts',(-20.5286666481821,-20.7775880208587,
-1.66567560158532));
#65101=CARTESIAN_POINT('Ctrl Pts',(-20.5888757444006,-20.7183987318922,
-1.66988536361091));
#65102=CARTESIAN_POINT('Ctrl Pts',(-20.6462548721938,-20.6561277358796,
-1.67409512563649));
#65103=CARTESIAN_POINT('Ctrl Pts',(-20.70047016696,-20.5910836105752,-1.67830488766208));
#65104=CARTESIAN_POINT('Ctrl Pts',(-20.7535207637169,-20.5274368172154,
-1.68242421208196));
#65105=CARTESIAN_POINT('Ctrl Pts',(-20.8035417749399,-20.4611352293305,
-1.68654353650185));
#65106=CARTESIAN_POINT('Ctrl Pts',(-20.8502568537434,-20.3925057892921,
-1.69066286092173));
#65107=CARTESIAN_POINT('Ctrl Pts',(-20.8969436352055,-20.3239179210705,
-1.69477969008884));
#65108=CARTESIAN_POINT('Ctrl Pts',(-20.940328192166,-20.2530053887166,-1.69889651925596));
#65109=CARTESIAN_POINT('Ctrl Pts',(-20.9801755792367,-20.1801267309364,
-1.70301334842307));
#65110=CARTESIAN_POINT('Ctrl Pts',(-21.0200115219931,-20.1072690041715,
-1.70712899522189));
#65111=CARTESIAN_POINT('Ctrl Pts',(-21.0563120854056,-20.0324466882332,
-1.71124464202071));
#65112=CARTESIAN_POINT('Ctrl Pts',(-21.0888874490411,-19.9560443726991,
-1.71536028881953));
#65113=CARTESIAN_POINT('Ctrl Pts',(-21.122756810271,-19.8766071129166,-1.71963942226786));
#65114=CARTESIAN_POINT('Ctrl Pts',(-21.1525985823987,-19.7954621912662,
-1.72391855571618));
#65115=CARTESIAN_POINT('Ctrl Pts',(-21.1782545829907,-19.7130647367531,
-1.7281976891645));
#65116=CARTESIAN_POINT('Ctrl Pts',(-21.2029529666689,-19.6337427887209,
-1.73231710284076));
#65117=CARTESIAN_POINT('Ctrl Pts',(-21.2237724306601,-19.5532606399815,
-1.73643651651702));
#65118=CARTESIAN_POINT('Ctrl Pts',(-21.2406233757609,-19.4720377410235,
-1.74055593019328));
#65119=CARTESIAN_POINT('Ctrl Pts',(-21.257483616485,-19.3907700364207,-1.74467761629503));
#65120=CARTESIAN_POINT('Ctrl Pts',(-21.2703709111432,-19.3087612356736,
-1.74879930239678));
#65121=CARTESIAN_POINT('Ctrl Pts',(-21.2792473404998,-19.2264375624415,
-1.75292098849853));
#65122=CARTESIAN_POINT('Ctrl Pts',(-21.2881358445687,-19.1440019033387,
-1.75704828137884));
#65123=CARTESIAN_POINT('Ctrl Pts',(-21.2930025792327,-19.061250988371,-1.76117557425916));
#65124=CARTESIAN_POINT('Ctrl Pts',(-21.2938616786583,-18.9786117668865,
-1.76530286713947));
#65125=CARTESIAN_POINT('Ctrl Pts',(-21.293959302996,-18.969221003687,-1.76577187482611));
#65126=CARTESIAN_POINT('Ctrl Pts',(-21.2940052315708,-18.95983167724,-1.76624088251274));
#65127=CARTESIAN_POINT('Ctrl Pts',(-21.2939995273704,-18.9504444089713,
-1.76670989019937));
#65128=CARTESIAN_POINT('Origin',(-18.734,-18.952,1.76670989022851));
#65129=CARTESIAN_POINT('',(-17.1769962711794,-16.9251779373085,-0.450077505597091));
#65130=CARTESIAN_POINT('',(-17.1722616763361,-16.9190322283098,-0.516748667021866));
#65131=CARTESIAN_POINT('',(-17.1744641548914,-16.9218650419685,1.76670989022851));
#65132=CARTESIAN_POINT('',(-21.2914666238416,-18.9551442278135,-0.166709890228505));
#65133=CARTESIAN_POINT('Ctrl Pts',(-21.2914666238416,-18.9551442278135,
-0.166709890228505));
#65134=CARTESIAN_POINT('Ctrl Pts',(-21.2869488473544,-18.3666789556461,
-0.195923797939959));
#65135=CARTESIAN_POINT('Ctrl Pts',(-20.7940986851072,-16.9152596074165,
-0.267529641211892));
#65136=CARTESIAN_POINT('Ctrl Pts',(-18.7954429923518,-16.112385634392,-0.361985513001419));
#65137=CARTESIAN_POINT('Ctrl Pts',(-17.5432453230646,-16.6451528738997,
-0.427227477079495));
#65138=CARTESIAN_POINT('Ctrl Pts',(-17.1769962711794,-16.9251779373085,
-0.450077505597091));
#65139=CARTESIAN_POINT('',(-19.3957372685685,-21.4249949024184,0.));
#65140=CARTESIAN_POINT('Ctrl Pts',(-19.3957372685684,-21.4249949024184,
8.32667268468867E-16));
#65141=CARTESIAN_POINT('Ctrl Pts',(-20.2191097516036,-21.2046724677036,
-0.0423919355604773));
#65142=CARTESIAN_POINT('Ctrl Pts',(-21.1334435320312,-20.3367930039316,
-0.0979618989699793));
#65143=CARTESIAN_POINT('Ctrl Pts',(-21.2935045362274,-19.2205935412502,
-0.153531862379481));
#65144=CARTESIAN_POINT('Ctrl Pts',(-21.2914666238416,-18.9551442278135,
-0.166709890228505));
#65145=CARTESIAN_POINT('',(-18.0722323438033,-21.4249867709335,-1.75387482315159E-11));
#65146=CARTESIAN_POINT('Origin',(-18.734,-18.952,0.));
#65147=CARTESIAN_POINT('',(-21.2939992553243,-18.9500473764188,-0.233290109771496));
#65148=CARTESIAN_POINT('Ctrl Pts',(-18.0722323438033,-21.4249867709335,
-1.75386372092134E-11));
#65149=CARTESIAN_POINT('Ctrl Pts',(-18.1529469590682,-21.4465858843588,
-0.0041815927697939));
#65150=CARTESIAN_POINT('Ctrl Pts',(-18.2348713083479,-21.4642696834585,
-0.00836318552204911));
#65151=CARTESIAN_POINT('Ctrl Pts',(-18.3175904330397,-21.4779063863382,
-0.0125447782743044));
#65152=CARTESIAN_POINT('Ctrl Pts',(-18.400191764092,-21.4915236702881,-0.0167204163572945));
#65153=CARTESIAN_POINT('Ctrl Pts',(-18.4835851718185,-21.5011052307698,
-0.0208960544402849));
#65154=CARTESIAN_POINT('Ctrl Pts',(-18.5673419980692,-21.5065694569521,
-0.025071692523275));
#65155=CARTESIAN_POINT('Ctrl Pts',(-18.6514951828607,-21.5120595412382,
-0.0292670907845262));
#65156=CARTESIAN_POINT('Ctrl Pts',(-18.7360147805747,-21.5133930942776,
-0.0334624890457766));
#65157=CARTESIAN_POINT('Ctrl Pts',(-18.8204570723937,-21.5105396566466,
-0.0376578873070279));
#65158=CARTESIAN_POINT('Ctrl Pts',(-18.9043499961556,-21.5077047830247,
-0.0418259909775909));
#65159=CARTESIAN_POINT('Ctrl Pts',(-18.9881661507819,-21.5007372505448,
-0.0459940946481546));
#65160=CARTESIAN_POINT('Ctrl Pts',(-19.0714685200795,-21.4896593541993,
-0.0501621983187175));
#65161=CARTESIAN_POINT('Ctrl Pts',(-19.1547428065988,-21.4785851924188,
-0.0543288968439942));
#65162=CARTESIAN_POINT('Ctrl Pts',(-19.2375031954147,-21.4634034794687,
-0.0584955953692703));
#65163=CARTESIAN_POINT('Ctrl Pts',(-19.3193181247986,-21.4441883341317,
-0.0626622938945471));
#65164=CARTESIAN_POINT('Ctrl Pts',(-19.4011301114166,-21.424973879936,-0.0668288425496348));
#65165=CARTESIAN_POINT('Ctrl Pts',(-19.4819962578844,-21.4017263881227,
-0.0709953912047227));
#65166=CARTESIAN_POINT('Ctrl Pts',(-19.5614968770271,-21.3745707251823,
-0.0751619398598105));
#65167=CARTESIAN_POINT('Ctrl Pts',(-19.6419526867073,-21.347088790163,-0.0793785491042684));
#65168=CARTESIAN_POINT('Ctrl Pts',(-19.72100947348,-21.3156042817862,-0.0835951583487267));
#65169=CARTESIAN_POINT('Ctrl Pts',(-19.7982514704289,-21.280297405335,-0.0878117675931847));
#65170=CARTESIAN_POINT('Ctrl Pts',(-19.8746836538425,-21.2453606900341,
-0.0919841694456243));
#65171=CARTESIAN_POINT('Ctrl Pts',(-19.9493385364599,-21.2066816487831,
-0.096156571298064));
#65172=CARTESIAN_POINT('Ctrl Pts',(-20.0218382563896,-21.1644811017,-0.100328973150504));
#65173=CARTESIAN_POINT('Ctrl Pts',(-20.0954901988232,-21.1216098703703,
-0.104567686090971));
#65174=CARTESIAN_POINT('Ctrl Pts',(-20.1669174627926,-21.0751044941558,
-0.108806399031438));
#65175=CARTESIAN_POINT('Ctrl Pts',(-20.2357562486613,-21.0252409820392,
-0.113045111971905));
#65176=CARTESIAN_POINT('Ctrl Pts',(-20.3045950345299,-20.9753774699226,
-0.117283824912372));
#65177=CARTESIAN_POINT('Ctrl Pts',(-20.3708449996543,-20.922156180229,-0.121522537852839));
#65178=CARTESIAN_POINT('Ctrl Pts',(-20.4341804646243,-20.8658929927532,
-0.125761250793306));
#65179=CARTESIAN_POINT('Ctrl Pts',(-20.4958618762422,-20.8110991607781,
-0.129889266554068));
#65180=CARTESIAN_POINT('Ctrl Pts',(-20.5550187782048,-20.7532072778741,
-0.13401728231483));
#65181=CARTESIAN_POINT('Ctrl Pts',(-20.6113174681947,-20.6924824399031,
-0.138145298075592));
#65182=CARTESIAN_POINT('Ctrl Pts',(-20.6675250873049,-20.6318558327154,
-0.142266636202703));
#65183=CARTESIAN_POINT('Ctrl Pts',(-20.7208833621661,-20.5684057202645,
-0.146387974329814));
#65184=CARTESIAN_POINT('Ctrl Pts',(-20.7710928145058,-20.5024363466744,
-0.150509312456925));
#65185=CARTESIAN_POINT('Ctrl Pts',(-20.8212566402015,-20.4365269211813,
-0.154626905416173));
#65186=CARTESIAN_POINT('Ctrl Pts',(-20.8682770342032,-20.36810315048,-0.158744498375422));
#65187=CARTESIAN_POINT('Ctrl Pts',(-20.9118931740675,-20.2975041145794,
-0.16286209133467));
#65188=CARTESIAN_POINT('Ctrl Pts',(-20.9554836015079,-20.2269466979588,
-0.166977256905893));
#65189=CARTESIAN_POINT('Ctrl Pts',(-20.9956735091388,-20.1542169629417,
-0.171092422477116));
#65190=CARTESIAN_POINT('Ctrl Pts',(-21.0322449112854,-20.0796836115466,
-0.17520758804834));
#65191=CARTESIAN_POINT('Ctrl Pts',(-21.0688064249755,-20.0051704130511,
-0.179321640929509));
#65192=CARTESIAN_POINT('Ctrl Pts',(-21.1017511684254,-19.9288549919469,
-0.183435693810678));
#65193=CARTESIAN_POINT('Ctrl Pts',(-21.1309074516109,-19.8511299507926,
-0.187549746691848));
#65194=CARTESIAN_POINT('Ctrl Pts',(-21.1600799699193,-19.7733616299242,
-0.19166609040528));
#65195=CARTESIAN_POINT('Ctrl Pts',(-21.1854596434762,-19.6941825637462,
-0.195782434118713));
#65196=CARTESIAN_POINT('Ctrl Pts',(-21.2069235785594,-19.6140037572439,
-0.199898777832145));
#65197=CARTESIAN_POINT('Ctrl Pts',(-21.2283934303839,-19.5338028486778,
-0.204016256255548));
#65198=CARTESIAN_POINT('Ctrl Pts',(-21.245945290129,-19.452602113539,-0.20813373467895));
#65199=CARTESIAN_POINT('Ctrl Pts',(-21.25950720014,-19.3708238078727,-0.212251213102353));
#65200=CARTESIAN_POINT('Ctrl Pts',(-21.2730871839159,-19.28893651742,-0.216374178830769));
#65201=CARTESIAN_POINT('Ctrl Pts',(-21.2826665420701,-19.2064705900184,
-0.220497144559185));
#65202=CARTESIAN_POINT('Ctrl Pts',(-21.2882251767647,-19.1238538518088,
-0.224620110287602));
#65203=CARTESIAN_POINT('Ctrl Pts',(-21.2921215111921,-19.0659435088809,
-0.227510110115567));
#65204=CARTESIAN_POINT('Ctrl Pts',(-21.2940434271759,-19.0079591563185,
-0.230400109943531));
#65205=CARTESIAN_POINT('Ctrl Pts',(-21.2939992553243,-18.9500473764188,
-0.233290109771496));
#65206=CARTESIAN_POINT('Ctrl Pts',(-21.2960080607363,-18.9500458442149,
-0.233290109771496));
#65207=CARTESIAN_POINT('Ctrl Pts',(-21.2971423972504,-18.8187089636245,
-0.239839092339242));
#65208=CARTESIAN_POINT('Ctrl Pts',(-21.2281784586555,-17.8383740905167,
-0.288780010467466));
#65209=CARTESIAN_POINT('Ctrl Pts',(-19.9618261937418,-16.1848209595297,
-0.380112864156168));
#65210=CARTESIAN_POINT('Ctrl Pts',(-17.9636855639766,-16.3488644542006,
-0.468050067338545));
#65211=CARTESIAN_POINT('Ctrl Pts',(-17.2221126135063,-16.8802618020223,
-0.513595334960445));
#65212=CARTESIAN_POINT('Ctrl Pts',(-17.1722616763361,-16.9190322283098,
-0.516748667021866));
#65213=CARTESIAN_POINT('Origin',(23.734,10.1295,-7.));
#65214=CARTESIAN_POINT('',(22.1191569089489,8.64088535679774,-10.9946458471364));
#65215=CARTESIAN_POINT('',(22.5286570306555,8.64088535511415,-10.994645846509));
#65216=CARTESIAN_POINT('',(23.734,8.64088535679774,-10.9946458471364));
#65217=CARTESIAN_POINT('',(23.534,7.33966741897454,-3.77664721604215));
#65218=CARTESIAN_POINT('Ctrl Pts',(23.534,7.33966741897454,-3.77664721604215));
#65219=CARTESIAN_POINT('Ctrl Pts',(23.51017627993,7.66133406205805,-3.49824266610593));
#65220=CARTESIAN_POINT('Ctrl Pts',(23.486909633093,8.02286895090474,-3.26954919204704));
#65221=CARTESIAN_POINT('Ctrl Pts',(23.4492315066612,8.63411569299029,-3.0005309807086));
#65222=CARTESIAN_POINT('Ctrl Pts',(23.4354446806246,8.8639010841975,-2.92198759519112));
#65223=CARTESIAN_POINT('Ctrl Pts',(23.399949158547,9.47603266342949,-2.76951143292666));
#65224=CARTESIAN_POINT('Ctrl Pts',(23.3787721949749,9.86402116292083,-2.72757919192478));
#65225=CARTESIAN_POINT('Ctrl Pts',(23.3407214533443,10.5425275171154,-2.747133164482));
#65226=CARTESIAN_POINT('Ctrl Pts',(23.3242429944554,10.8311360244973,-2.78512529399453));
#65227=CARTESIAN_POINT('Ctrl Pts',(23.2929661635979,11.3716051953523,-2.91335793594839));
#65228=CARTESIAN_POINT('Ctrl Pts',(23.2783733783153,11.6233081664386,-2.99849923355931));
#65229=CARTESIAN_POINT('Ctrl Pts',(23.2328152819286,12.3725180640175,-3.33254296279843));
#65230=CARTESIAN_POINT('Ctrl Pts',(23.2012866427256,12.8305461368956,-3.65549380921278));
#65231=CARTESIAN_POINT('Ctrl Pts',(23.1549367702088,13.4067359697088,-4.25937645462649));
#65232=CARTESIAN_POINT('Ctrl Pts',(23.1395239514397,13.5793277462794,-4.48008348661314));
#65233=CARTESIAN_POINT('Ctrl Pts',(23.1099688138179,13.8617277895674,-4.92516171922708));
#65234=CARTESIAN_POINT('Ctrl Pts',(23.0959457347052,13.9759147216023,-5.14539286840817));
#65235=CARTESIAN_POINT('Ctrl Pts',(23.0504578182471,14.2830486657584,-5.88990281436943));
#65236=CARTESIAN_POINT('Ctrl Pts',(23.0202677929568,14.3925081775317,-6.44228728766363));
#65237=CARTESIAN_POINT('Ctrl Pts',(22.9756095483293,14.39249658211,-7.23314652577812));
#65238=CARTESIAN_POINT('Ctrl Pts',(22.9623778488159,14.3733770772517,-7.46584216670397));
#65239=CARTESIAN_POINT('Ctrl Pts',(22.9358798283986,14.2959926399339,-7.93359342777265));
#65240=CARTESIAN_POINT('Ctrl Pts',(22.9226192672182,14.2365591328009,-8.16761560319146));
#65241=CARTESIAN_POINT('Ctrl Pts',(22.8884454080608,14.0354961954562,-8.7480497067035));
#65242=CARTESIAN_POINT('Ctrl Pts',(22.867361205658,13.8675338973621,-9.08316268713324));
#65243=CARTESIAN_POINT('Ctrl Pts',(22.83129324382,13.5087614903736,-9.61239330323816));
#65244=CARTESIAN_POINT('Ctrl Pts',(22.816606886244,13.3391139157858,-9.81822440975084));
#65245=CARTESIAN_POINT('Ctrl Pts',(22.7763959093789,12.8279581857622,-10.3319271922136));
#65246=CARTESIAN_POINT('Ctrl Pts',(22.7505181760814,12.4542070728383,-10.6026540019325));
#65247=CARTESIAN_POINT('Ctrl Pts',(22.6994595055266,11.6432335511213,-11.0104357195506));
#65248=CARTESIAN_POINT('Ctrl Pts',(22.6750357731946,11.2124938682904,-11.1475429363853));
#65249=CARTESIAN_POINT('Ctrl Pts',(22.6356443648331,10.5204537580763,-11.2524316658375));
#65250=CARTESIAN_POINT('Ctrl Pts',(22.6214072895926,10.2697555020984,-11.2680612232353));
#65251=CARTESIAN_POINT('Ctrl Pts',(22.5828683772762,9.58434848171878,-11.2503118781594));
#65252=CARTESIAN_POINT('Ctrl Pts',(22.5592032550112,9.15383198149799,-11.1725793563088));
#65253=CARTESIAN_POINT('Ctrl Pts',(22.5327132940792,8.70849794314267,-11.0193555381541));
#65254=CARTESIAN_POINT('Ctrl Pts',(22.5306859582416,8.67460721925019,-11.007212382501));
#65255=CARTESIAN_POINT('Ctrl Pts',(22.5286570306555,8.64088535511415,-10.994645846509));
#65256=CARTESIAN_POINT('',(23.533999981869,7.33961491412,-10.2235360410646));
#65257=CARTESIAN_POINT('Origin',(23.534,10.1295,-7.));
#65258=CARTESIAN_POINT('',(22.2043183294109,10.1294634651143,-11.262893868652));
#65259=CARTESIAN_POINT('Ctrl Pts',(23.533999981869,7.33961491412,-10.2235360410646));
#65260=CARTESIAN_POINT('Ctrl Pts',(23.5009788547464,6.89416391178422,-9.83730563779938));
#65261=CARTESIAN_POINT('Ctrl Pts',(23.4291758459878,6.10016038128925,-8.79502345374906));
#65262=CARTESIAN_POINT('Ctrl Pts',(23.3185909555934,5.6985094017683,-6.80076298606476));
#65263=CARTESIAN_POINT('Ctrl Pts',(23.2022453106851,6.3076790998453,-4.74899581907506));
#65264=CARTESIAN_POINT('Ctrl Pts',(23.085899665777,7.80672899094502,-3.22136567669558));
#65265=CARTESIAN_POINT('Ctrl Pts',(22.9695540208687,9.84662493401956,-2.57356512891912));
#65266=CARTESIAN_POINT('Ctrl Pts',(22.8532083759605,11.9523856169729,-2.95643327596383));
#65267=CARTESIAN_POINT('Ctrl Pts',(22.7368627310523,13.6336979697146,-4.28082124831138));
#65268=CARTESIAN_POINT('Ctrl Pts',(22.6205170861441,14.4990821903827,-6.2383517396752));
#65269=CARTESIAN_POINT('Ctrl Pts',(22.5041714412359,14.3470299002299,-8.3732307562808));
#65270=CARTESIAN_POINT('Ctrl Pts',(22.3878257963277,13.2129653049274,-10.1883541012585));
#65271=CARTESIAN_POINT('Ctrl Pts',(22.2878747590527,11.6218855899156,-11.109940009747));
#65272=CARTESIAN_POINT('Ctrl Pts',(22.2267056034138,10.5292997601409,-11.262549287517));
#65273=CARTESIAN_POINT('Ctrl Pts',(22.2043183294109,10.1294634667828,-11.26269919276));
#65274=CARTESIAN_POINT('Ctrl Pts',(22.2043183294109,10.1294634642048,-11.2629999998434));
#65275=CARTESIAN_POINT('Ctrl Pts',(22.1969189590874,9.99730152393924,-11.2629988671572));
#65276=CARTESIAN_POINT('Ctrl Pts',(22.189519588764,9.86515952805542,-11.2568474502169));
#65277=CARTESIAN_POINT('Ctrl Pts',(22.1821202184405,9.73360519517336,-11.2445772820755));
#65278=CARTESIAN_POINT('Ctrl Pts',(22.174718676944,9.60201226073271,-11.2323035135386));
#65279=CARTESIAN_POINT('Ctrl Pts',(22.1673171354475,9.47100764621991,-11.2139074381013));
#65280=CARTESIAN_POINT('Ctrl Pts',(22.1599155939509,9.34115385194522,-11.1894724430228));
#65281=CARTESIAN_POINT('Ctrl Pts',(22.1583218981377,9.31319380492507,-11.184211113424));
#65282=CARTESIAN_POINT('Ctrl Pts',(22.1567282023245,9.28528708178846,-11.1786699942205));
#65283=CARTESIAN_POINT('Ctrl Pts',(22.1551345065113,9.25743924154366,-11.1728502289874));
#65284=CARTESIAN_POINT('Ctrl Pts',(22.147885780794,9.1307768295063,-11.1463797560378));
#65285=CARTESIAN_POINT('Ctrl Pts',(22.1406370550766,9.00529749216246,-11.1141331631283));
#65286=CARTESIAN_POINT('Ctrl Pts',(22.1333883293593,8.8815309348635,-11.0762411867384));
#65287=CARTESIAN_POINT('Ctrl Pts',(22.1286445225558,8.80053399009637,-11.0514434191851));
#65288=CARTESIAN_POINT('Ctrl Pts',(22.1239007157524,8.7202703940275,-11.0242288773707));
#65289=CARTESIAN_POINT('Ctrl Pts',(22.1191569089489,8.64088535679774,-10.9946458471364));
#65290=CARTESIAN_POINT('Origin',(23.734,10.1295,-7.));
#65291=CARTESIAN_POINT('',(20.6190482080202,8.64088535679775,-10.9946458471364));
#65292=CARTESIAN_POINT('',(21.0285562485163,8.64088535679775,-10.9946458471364));
#65293=CARTESIAN_POINT('',(23.734,8.64088535679774,-10.9946458471364));
#65294=CARTESIAN_POINT('',(21.113681670589,10.1298201264287,-11.2629999879802));
#65295=CARTESIAN_POINT('Ctrl Pts',(21.0285562485163,8.64088535679774,-10.9946458471364));
#65296=CARTESIAN_POINT('Ctrl Pts',(21.0355842654606,8.75858542230884,-11.0385070673122));
#65297=CARTESIAN_POINT('Ctrl Pts',(21.042612282405,8.878246078405,-11.0771699233389));
#65298=CARTESIAN_POINT('Ctrl Pts',(21.0496402993493,8.99937754862533,-11.1104734818387));
#65299=CARTESIAN_POINT('Ctrl Pts',(21.0566702577254,9.12054248041531,-11.1437862401718));
#65300=CARTESIAN_POINT('Ctrl Pts',(21.0637002161014,9.24317866806857,-11.1717366365414));
#65301=CARTESIAN_POINT('Ctrl Pts',(21.0707301744775,9.36678222315231,-11.1942139421923));
#65302=CARTESIAN_POINT('Ctrl Pts',(21.0774006019609,9.48406436150666,-11.215541698254));
#65303=CARTESIAN_POINT('Ctrl Pts',(21.0840710294444,9.60221707186205,-11.2319422034653));
#65304=CARTESIAN_POINT('Ctrl Pts',(21.0907414569279,9.7208031090756,-11.2433637425218));
#65305=CARTESIAN_POINT('Ctrl Pts',(21.0983881948149,9.8567458722469,-11.2564569836444));
#65306=CARTESIAN_POINT('Ctrl Pts',(21.106034932702,9.99328288766813,-11.2630102411303));
#65307=CARTESIAN_POINT('Ctrl Pts',(21.113681670589,10.1298201264287,-11.2629999879802));
#65308=CARTESIAN_POINT('Ctrl Pts',(22.5286570306555,8.64088535511415,-10.994645846509));
#65309=CARTESIAN_POINT('Ctrl Pts',(22.5118636558758,8.36177046378126,-10.8906329926018));
#65310=CARTESIAN_POINT('Ctrl Pts',(22.4949371726258,8.09422513235076,-10.7576155574016));
#65311=CARTESIAN_POINT('Ctrl Pts',(22.4658689060726,7.65365862514857,-10.4775761889738));
#65312=CARTESIAN_POINT('Ctrl Pts',(22.4535279654699,7.47441140277351,-10.3427282621983));
#65313=CARTESIAN_POINT('Ctrl Pts',(22.4257237608203,7.10029198315386,-10.0121190423));
#65314=CARTESIAN_POINT('Ctrl Pts',(22.4102377872913,6.9121452084373,-9.81026367361129));
#65315=CARTESIAN_POINT('Ctrl Pts',(22.3707645547773,6.48795081170686,-9.25627062175758));
#65316=CARTESIAN_POINT('Ctrl Pts',(22.3475332522488,6.28239420355209,-8.88452324880333));
#65317=CARTESIAN_POINT('Ctrl Pts',(22.2991968287437,5.97938706676746,-8.07143465124029));
#65318=CARTESIAN_POINT('Ctrl Pts',(22.273851585444,5.89022879368264,-7.63244016957764));
#65319=CARTESIAN_POINT('Ctrl Pts',(22.2344146536939,5.85912002685203,-6.9263610284236));
#65320=CARTESIAN_POINT('Ctrl Pts',(22.2200353762392,5.87167646499845,-6.66457609220379));
#65321=CARTESIAN_POINT('Ctrl Pts',(22.1818223710797,5.96723863349493,-5.98591179105523));
#65322=CARTESIAN_POINT('Ctrl Pts',(22.1576958095408,6.08858787963603,-5.57739186590976));
#65323=CARTESIAN_POINT('Ctrl Pts',(22.1205062536004,6.37074684053622,-4.97428398518268));
#65324=CARTESIAN_POINT('Ctrl Pts',(22.1071894019662,6.49179727944132,-4.76418413843906));
#65325=CARTESIAN_POINT('Ctrl Pts',(22.0671850918357,6.90229670185062,-4.17411268177498));
#65326=CARTESIAN_POINT('Ctrl Pts',(22.0400473276349,7.23830147516879,-3.83117576454053));
#65327=CARTESIAN_POINT('Ctrl Pts',(21.9977748536775,7.85232129043855,-3.38513612330148));
#65328=CARTESIAN_POINT('Ctrl Pts',(21.9822603591102,8.0965069728334,-3.24237784686094));
#65329=CARTESIAN_POINT('Ctrl Pts',(21.9508581575842,8.6070684025483,-3.0083229022697));
#65330=CARTESIAN_POINT('Ctrl Pts',(21.9350483246724,8.87196946541536,-2.91712190086957));
#65331=CARTESIAN_POINT('Ctrl Pts',(21.8879430145404,9.68327455895831,-2.72432043907536));
#65332=CARTESIAN_POINT('Ctrl Pts',(21.8579319608022,10.2425282684304,-2.70258470449789));
#65333=CARTESIAN_POINT('Ctrl Pts',(21.8116740680761,11.0520540128713,-2.82959340678504));
#65334=CARTESIAN_POINT('Ctrl Pts',(21.7966310224467,11.3094654254284,-2.89499238840428));
#65335=CARTESIAN_POINT('Ctrl Pts',(21.7656906411665,11.8324564954503,-3.08116396146755));
#65336=CARTESIAN_POINT('Ctrl Pts',(21.7497498339434,12.0951273402525,-3.20610388733662));
#65337=CARTESIAN_POINT('Ctrl Pts',(21.7178985270123,12.5819652847213,-3.50189737230709));
#65338=CARTESIAN_POINT('Ctrl Pts',(21.7020850761519,12.8060015909147,-3.67018921888465));
#65339=CARTESIAN_POINT('Ctrl Pts',(21.6554218096547,13.414664248813,-4.22878178565749));
#65340=CARTESIAN_POINT('Ctrl Pts',(21.6258177033332,13.7425641809248,-4.672399799817));
#65341=CARTESIAN_POINT('Ctrl Pts',(21.5800184528173,14.091699551123,-5.40491681528636));
#65342=CARTESIAN_POINT('Ctrl Pts',(21.5649766711582,14.1831276533754,-5.65410747919475));
#65343=CARTESIAN_POINT('Ctrl Pts',(21.5244527242273,14.3689368074488,-6.35677233692095));
#65344=CARTESIAN_POINT('Ctrl Pts',(21.4991530720328,14.4136600195989,-6.81960777591371));
#65345=CARTESIAN_POINT('Ctrl Pts',(21.4579890825941,14.3657168863367,-7.54651079827598));
#65346=CARTESIAN_POINT('Ctrl Pts',(21.4429061062594,14.3232719350075,-7.81024381229356));
#65347=CARTESIAN_POINT('Ctrl Pts',(21.4159048305994,14.2016669275244,-8.28002389107006));
#65348=CARTESIAN_POINT('Ctrl Pts',(21.4038280841489,14.1306451549211,-8.48722632324378));
#65349=CARTESIAN_POINT('Ctrl Pts',(21.3837784855311,13.9883604529451,-8.81717803075001));
#65350=CARTESIAN_POINT('Ctrl Pts',(21.3758969361811,13.9263289765945,-8.94345786773658));
#65351=CARTESIAN_POINT('Ctrl Pts',(21.3539492458001,13.7375378316432,-9.28411162819851));
#65352=CARTESIAN_POINT('Ctrl Pts',(21.3398129173365,13.5980747677776,-9.49080140356762));
#65353=CARTESIAN_POINT('Ctrl Pts',(21.3135714918117,13.3034777608084,-9.85429566101133));
#65354=CARTESIAN_POINT('Ctrl Pts',(21.3015202725534,13.1526673276748,-10.0135693682859));
#65355=CARTESIAN_POINT('Ctrl Pts',(21.2602281400547,12.5999537871976,-10.5138599540741));
#65356=CARTESIAN_POINT('Ctrl Pts',(21.2303768190197,12.1475356841319,-10.7918148242534));
#65357=CARTESIAN_POINT('Ctrl Pts',(21.1865848300647,11.4157097369092,-11.0724755597816));
#65358=CARTESIAN_POINT('Ctrl Pts',(21.1723949368264,11.167582150591,-11.1426779064966));
#65359=CARTESIAN_POINT('Ctrl Pts',(21.1433266163339,10.6558371681204,-11.2385692421312));
#65360=CARTESIAN_POINT('Ctrl Pts',(21.1284972322154,10.3931077210865,-11.2629799952814));
#65361=CARTESIAN_POINT('Ctrl Pts',(21.1136182667127,10.1298237102038,-11.2629999877096));
#65362=CARTESIAN_POINT('',(20.7043183293681,10.1330470781642,-11.2629985243062));
#65363=CARTESIAN_POINT('Ctrl Pts',(22.1191569089489,8.64088535679774,-10.9946458471364));
#65364=CARTESIAN_POINT('Ctrl Pts',(22.1119092550574,8.5195997948344,-10.9494484828501));
#65365=CARTESIAN_POINT('Ctrl Pts',(22.1046616011658,8.40036603378345,-10.8987202994482));
#65366=CARTESIAN_POINT('Ctrl Pts',(22.0974139472743,8.28368678979871,-10.8426738858569));
#65367=CARTESIAN_POINT('Ctrl Pts',(22.0901668484829,8.16701648231366,-10.7866317648778));
#65368=CARTESIAN_POINT('Ctrl Pts',(22.0829197496915,8.05290061237157,-10.7252723788802));
#65369=CARTESIAN_POINT('Ctrl Pts',(22.0756726509,7.94181920681921,-10.6588552509149));
#65370=CARTESIAN_POINT('Ctrl Pts',(22.0684237902754,7.83071079640412,-10.5924219763641));
#65371=CARTESIAN_POINT('Ctrl Pts',(22.0611749296508,7.72263862195278,-10.5209286802897));
#65372=CARTESIAN_POINT('Ctrl Pts',(22.0539260690261,7.61805591081906,-10.4446796058441));
#65373=CARTESIAN_POINT('Ctrl Pts',(22.0488803332185,7.54525871443813,-10.3916046875702));
#65374=CARTESIAN_POINT('Ctrl Pts',(22.0438345974108,7.47415165964849,-10.3362264444816));
#65375=CARTESIAN_POINT('Ctrl Pts',(22.0387888616031,7.40487871978231,-10.2786594637725));
#65376=CARTESIAN_POINT('Ctrl Pts',(22.0315394209714,7.30535110199038,-10.1959503357274));
#65377=CARTESIAN_POINT('Ctrl Pts',(22.0242899803397,7.20957401612299,-10.1086907026288));
#65378=CARTESIAN_POINT('Ctrl Pts',(22.017040539708,7.11795438636582,-10.0172441096141));
#65379=CARTESIAN_POINT('Ctrl Pts',(22.0097925532381,7.02635313454589,-9.9258158598272));
#65380=CARTESIAN_POINT('Ctrl Pts',(22.0025445667682,6.93890792009219,-9.83020256976117));
#65381=CARTESIAN_POINT('Ctrl Pts',(21.9952965802982,6.85598915380836,-9.73080496188683));
#65382=CARTESIAN_POINT('Ctrl Pts',(21.9880483796479,6.77306793724778,-9.63140441678055));
#65383=CARTESIAN_POINT('Ctrl Pts',(21.9808001789976,6.6946736606481,-9.52821959371692));
#65384=CARTESIAN_POINT('Ctrl Pts',(21.9735519783473,6.62113693951177,-9.4216848754125));
#65385=CARTESIAN_POINT('Ctrl Pts',(21.9663041219354,6.54760371085093,-9.31515521675567));
#65386=CARTESIAN_POINT('Ctrl Pts',(21.9590562655235,6.47892777135004,-9.2052762668258));
#65387=CARTESIAN_POINT('Ctrl Pts',(21.9518084091116,6.41539671901929,-9.09251184422175));
#65388=CARTESIAN_POINT('Ctrl Pts',(21.9445590323088,6.35185233970911,-8.97972376689949));
#65389=CARTESIAN_POINT('Ctrl Pts',(21.937309655506,6.29345517258953,-8.86404930972801));
#65390=CARTESIAN_POINT('Ctrl Pts',(21.9300602787033,6.24044729171331,-8.74597767229939));
#65391=CARTESIAN_POINT('Ctrl Pts',(21.9275212580338,6.22188181928044,-8.70462427930291));
#65392=CARTESIAN_POINT('Ctrl Pts',(21.9249822373644,6.20397701830355,-8.66297703249341));
#65393=CARTESIAN_POINT('Ctrl Pts',(21.922443216695,6.18674190960378,-8.62105756856911));
#65394=CARTESIAN_POINT('Ctrl Pts',(21.9151754459718,6.13740760526893,-8.50106600792267));
#65395=CARTESIAN_POINT('Ctrl Pts',(21.9079076752487,6.09354713243275,-8.37880167535367));
#65396=CARTESIAN_POINT('Ctrl Pts',(21.9006399045255,6.05534999136786,-8.25477914676757));
#65397=CARTESIAN_POINT('Ctrl Pts',(21.8933734613687,6.01715982757829,-8.13077927273893));
#65398=CARTESIAN_POINT('Ctrl Pts',(21.8861070182118,5.98463103242785,-8.00502217048947));
#65399=CARTESIAN_POINT('Ctrl Pts',(21.878840575055,5.95790341045558,-7.87803809376438));
#65400=CARTESIAN_POINT('Ctrl Pts',(21.871573922425,5.93117501799356,-7.75105035640947));
#65401=CARTESIAN_POINT('Ctrl Pts',(21.8643072697949,5.91024820677359,-7.6228359082289));
#65402=CARTESIAN_POINT('Ctrl Pts',(21.8570406171649,5.89521184619667,-7.49393605918256));
#65403=CARTESIAN_POINT('Ctrl Pts',(21.8497743641547,5.8801763125242,-7.36504329881022));
#65404=CARTESIAN_POINT('Ctrl Pts',(21.8425081111445,5.8710306198732,-7.23546555319564));
#65405=CARTESIAN_POINT('Ctrl Pts',(21.8352418581342,5.86781184389181,-7.10574998859196));
#65406=CARTESIAN_POINT('Ctrl Pts',(21.8279743223649,5.8645924996789,-6.9760115244532));
#65407=CARTESIAN_POINT('Ctrl Pts',(21.8207067865956,5.86730217015556,-6.84613553506541));
#65408=CARTESIAN_POINT('Ctrl Pts',(21.8134392508263,5.87592582273696,-6.7166703006725));
#65409=CARTESIAN_POINT('Ctrl Pts',(21.8109920244798,5.878829699714,-6.67307495520454));
#65410=CARTESIAN_POINT('Ctrl Pts',(21.8085447981333,5.88240372517832,-6.62952616917805));
#65411=CARTESIAN_POINT('Ctrl Pts',(21.8060975717868,5.88664599746917,-6.58604479323473));
#65412=CARTESIAN_POINT('Ctrl Pts',(21.7989003324876,5.89912242773205,-6.45816701512477));
#65413=CARTESIAN_POINT('Ctrl Pts',(21.7917030931884,5.9173874845122,-6.33082262933598));
#65414=CARTESIAN_POINT('Ctrl Pts',(21.7845058538891,5.94137144353383,-6.20454529072198));
#65415=CARTESIAN_POINT('Ctrl Pts',(21.777310240048,5.96534998590645,-6.07829647117027));
#65416=CARTESIAN_POINT('Ctrl Pts',(21.7701146262068,5.9950447885472,-5.95311456770553));
#65417=CARTESIAN_POINT('Ctrl Pts',(21.7629190123656,6.03033483538351,-5.82952404843386));
#65418=CARTESIAN_POINT('Ctrl Pts',(21.7557229447161,6.06562710786945,-5.705925734636));
#65419=CARTESIAN_POINT('Ctrl Pts',(21.7485268770667,6.10651523595494,-5.58391934900157));
#65420=CARTESIAN_POINT('Ctrl Pts',(21.7413308094172,6.15282797750728,-5.46401542145645));
#65421=CARTESIAN_POINT('Ctrl Pts',(21.7341348236115,6.199140192326,-5.34411285762736));
#65422=CARTESIAN_POINT('Ctrl Pts',(21.7269388378059,6.25087676563492,-5.22631303483247));
#65423=CARTESIAN_POINT('Ctrl Pts',(21.7197428520002,6.3078179577087,-5.11110737001062));
#65424=CARTESIAN_POINT('Ctrl Pts',(21.7125445442252,6.36477752331817,-4.99586453112694));
#65425=CARTESIAN_POINT('Ctrl Pts',(21.7053462364502,6.42694490292231,-4.88321784067244));
#65426=CARTESIAN_POINT('Ctrl Pts',(21.6981479286752,6.49405382499079,-4.77363522561758));
#65427=CARTESIAN_POINT('Ctrl Pts',(21.6953492614097,6.52014544947959,-4.73103003461787));
#65428=CARTESIAN_POINT('Ctrl Pts',(21.6925505941441,6.54698356415018,-4.68888773294117));
#65429=CARTESIAN_POINT('Ctrl Pts',(21.6897519268785,6.57455071884714,-4.64723468904552));
#65430=CARTESIAN_POINT('Ctrl Pts',(21.6823654767811,6.64730799692895,-4.53730088807892));
#65431=CARTESIAN_POINT('Ctrl Pts',(21.6749790266836,6.72517120219222,-4.43074005094906));
#65432=CARTESIAN_POINT('Ctrl Pts',(21.6675925765861,6.8078078071312,-4.32801010933154));
#65433=CARTESIAN_POINT('Ctrl Pts',(21.6602070407686,6.89043418347741,-4.22529288341958));
#65434=CARTESIAN_POINT('Ctrl Pts',(21.652821504951,6.97783258068516,-4.12640585384117));
#65435=CARTESIAN_POINT('Ctrl Pts',(21.6454359691335,7.06962978046818,-4.03177439543045));
#65436=CARTESIAN_POINT('Ctrl Pts',(21.6380510733541,7.16141902501109,-3.93715113787961));
#65437=CARTESIAN_POINT('Ctrl Pts',(21.6306661775747,7.2576060910435,-3.84678294446063));
#65438=CARTESIAN_POINT('Ctrl Pts',(21.6232812817953,7.3577801678109,-3.76105909719711));
#65439=CARTESIAN_POINT('Ctrl Pts',(21.6158977417591,7.45793585429648,-3.67535098739542));
#65440=CARTESIAN_POINT('Ctrl Pts',(21.6085142017228,7.56207684856391,-3.59428572780241));
#65441=CARTESIAN_POINT('Ctrl Pts',(21.6011306616865,7.66975832511667,-3.51821311783129));
#65442=CARTESIAN_POINT('Ctrl Pts',(21.5937483307954,7.77742216750874,-3.4421529656818));
#65443=CARTESIAN_POINT('Ctrl Pts',(21.5863659999042,7.88862507567842,-3.3710840148624));
#65444=CARTESIAN_POINT('Ctrl Pts',(21.5789836690131,8.0028919322252,-3.30531366337072));
#65445=CARTESIAN_POINT('Ctrl Pts',(21.5771245399989,8.03166832162039,-3.28875038944878));
#65446=CARTESIAN_POINT('Ctrl Pts',(21.5752654109847,8.06063888910807,-3.27252294045707));
#65447=CARTESIAN_POINT('Ctrl Pts',(21.5734062819705,8.08979577177236,-3.25663578296871));
#65448=CARTESIAN_POINT('Ctrl Pts',(21.5663766750943,8.20004171021903,-3.19656438896128));
#65449=CARTESIAN_POINT('Ctrl Pts',(21.5593470682181,8.31298831198066,-3.14134266250149));
#65450=CARTESIAN_POINT('Ctrl Pts',(21.5523174613419,8.42817722338396,-3.0912060926972));
#65451=CARTESIAN_POINT('Ctrl Pts',(21.5452896275042,8.54333708133278,-3.04108216855934));
#65452=CARTESIAN_POINT('Ctrl Pts',(21.5382617936664,8.6607377697407,-2.99604099920424));
#65453=CARTESIAN_POINT('Ctrl Pts',(21.5312339598286,8.7798993723283,-2.95627063890421));
#65454=CARTESIAN_POINT('Ctrl Pts',(21.5242047012697,8.89908513201198,-2.9164922161378));
#65455=CARTESIAN_POINT('Ctrl Pts',(21.5171754427108,9.02003215567398,-2.88198686387374));
#65456=CARTESIAN_POINT('Ctrl Pts',(21.5101461841518,9.14224366034339,-2.85289330739999));
#65457=CARTESIAN_POINT('Ctrl Pts',(21.5031162567188,9.26446679413621,-2.82379698250799));
#65458=CARTESIAN_POINT('Ctrl Pts',(21.4960863292857,9.38795427288864,-2.80011356232756));
#65459=CARTESIAN_POINT('Ctrl Pts',(21.4890564018526,9.5121981594764,-2.78193084010158));
#65460=CARTESIAN_POINT('Ctrl Pts',(21.4820218975376,9.63652293588892,-2.76373627989101));
#65461=CARTESIAN_POINT('Ctrl Pts',(21.4749873932226,9.76160472207926,-2.75104962078328));
#65462=CARTESIAN_POINT('Ctrl Pts',(21.4679528889076,9.88692926940032,-2.74390690413657));
#65463=CARTESIAN_POINT('Ctrl Pts',(21.4643221382925,9.95161359638359,-2.74022030139992));
#65464=CARTESIAN_POINT('Ctrl Pts',(21.4606913876774,10.0163625427089,-2.73800972683479));
#65465=CARTESIAN_POINT('Ctrl Pts',(21.4570606370622,10.0811053611285,-2.737274702854));
#65466=CARTESIAN_POINT('Ctrl Pts',(21.4494491623812,10.216831654508,-2.73573380483792));
#65467=CARTESIAN_POINT('Ctrl Pts',(21.4418376877003,10.3526182676046,-2.74067973952619));
#65468=CARTESIAN_POINT('Ctrl Pts',(21.4342262130193,10.4878649307102,-2.75208950465796));
#65469=CARTESIAN_POINT('Ctrl Pts',(21.4264336112805,10.6263300017054,-2.76377078316592));
#65470=CARTESIAN_POINT('Ctrl Pts',(21.4186410095417,10.764228814435,-2.78222738393882));
#65471=CARTESIAN_POINT('Ctrl Pts',(21.410848407803,10.9009217006177,-2.80737819976378));
#65472=CARTESIAN_POINT('Ctrl Pts',(21.4032429171247,11.0343324030374,-2.83192510998959));
#65473=CARTESIAN_POINT('Ctrl Pts',(21.3956374264465,11.1665941568544,-2.86284837110384));
#65474=CARTESIAN_POINT('Ctrl Pts',(21.3880319357682,11.2971204731094,-2.90002055727401));
#65475=CARTESIAN_POINT('Ctrl Pts',(21.3801457784992,11.4324636220633,-2.93856451434043));
#65476=CARTESIAN_POINT('Ctrl Pts',(21.3722596212301,11.5659405054026,-2.98382740162559));
#65477=CARTESIAN_POINT('Ctrl Pts',(21.3643734639611,11.6969110187463,-3.03560954265189));
#65478=CARTESIAN_POINT('Ctrl Pts',(21.3564873066921,11.8278815320899,-3.08739168367819));
#65479=CARTESIAN_POINT('Ctrl Pts',(21.3486011494231,11.956345363596,-3.14569299962129));
#65480=CARTESIAN_POINT('Ctrl Pts',(21.340714992154,12.0816810369674,-3.21025618294525));
#65481=CARTESIAN_POINT('Ctrl Pts',(21.3336759604758,12.1935532384943,-3.26788403351437));
#65482=CARTESIAN_POINT('Ctrl Pts',(21.3266369287976,12.3028932792345,-3.33048051016728));
#65483=CARTESIAN_POINT('Ctrl Pts',(21.3195978971194,12.40925055225,-3.39779145252306));
#65484=CARTESIAN_POINT('Ctrl Pts',(21.3125590744663,12.5156046669697,-3.46510039606998));
#65485=CARTESIAN_POINT('Ctrl Pts',(21.3055202518132,12.6189758680056,-3.53712332086819));
#65486=CARTESIAN_POINT('Ctrl Pts',(21.2984814291601,12.7189414344944,-3.61356203994173));
#65487=CARTESIAN_POINT('Ctrl Pts',(21.2914389136867,12.8189594465259,-3.69004086152499));
#65488=CARTESIAN_POINT('Ctrl Pts',(21.2843963982133,12.9155679496317,-3.77093987410838));
#65489=CARTESIAN_POINT('Ctrl Pts',(21.2773538827399,13.0083761165701,-3.85591964074671));
#65490=CARTESIAN_POINT('Ctrl Pts',(21.2703094098651,13.1012100786724,-3.94092302671816));
#65491=CARTESIAN_POINT('Ctrl Pts',(21.2632649369902,13.1902413235328,-4.03000916216276));
#65492=CARTESIAN_POINT('Ctrl Pts',(21.2562204641154,13.2751155328051,-4.12280137637754));
#65493=CARTESIAN_POINT('Ctrl Pts',(21.2491695588495,13.3600672417159,-4.21567832025411));
#65494=CARTESIAN_POINT('Ctrl Pts',(21.2421186535837,13.4408540813723,-4.31226781405213));
#65495=CARTESIAN_POINT('Ctrl Pts',(21.2350677483178,13.5171614727389,-4.41215944345081));
#65496=CARTESIAN_POINT('Ctrl Pts',(21.2315016146271,13.5557554332217,-4.46268159508693));
#65497=CARTESIAN_POINT('Ctrl Pts',(21.2279354809365,13.5932042061302,-4.51404795176234));
#65498=CARTESIAN_POINT('Ctrl Pts',(21.2243693472458,13.6294713302574,-4.56620261990112));
#65499=CARTESIAN_POINT('Ctrl Pts',(21.2173459273525,13.7008986134619,-4.66892006279847));
#65500=CARTESIAN_POINT('Ctrl Pts',(21.2103225074592,13.7678679518273,-4.77488136034603));
#65501=CARTESIAN_POINT('Ctrl Pts',(21.2032990875659,13.8300824556287,-4.88366862493296));
#65502=CARTESIAN_POINT('Ctrl Pts',(21.1962814937663,13.8922453510204,-4.99236564789809));
#65503=CARTESIAN_POINT('Ctrl Pts',(21.1892638999668,13.9496610740247,-5.10388363594717));
#65504=CARTESIAN_POINT('Ctrl Pts',(21.1822463061672,14.0020763560252,-5.21777628599693));
#65505=CARTESIAN_POINT('Ctrl Pts',(21.1752329695233,14.0544598407996,-5.33159984416752));
#65506=CARTESIAN_POINT('Ctrl Pts',(21.1682196328795,14.1018487643949,-5.44779484503741));
#65507=CARTESIAN_POINT('Ctrl Pts',(21.1612062962356,14.1440362326073,-5.5658912743158));
#65508=CARTESIAN_POINT('Ctrl Pts',(21.1541426196187,14.1865265118952,-5.68483537017137));
#65509=CARTESIAN_POINT('Ctrl Pts',(21.1470789430017,14.223740187332,-5.80570794539113));
#65510=CARTESIAN_POINT('Ctrl Pts',(21.1400152663848,14.2555155490246,-5.92800900693764));
#65511=CARTESIAN_POINT('Ctrl Pts',(21.1330043158592,14.2870537267815,-6.04939716472518));
#65512=CARTESIAN_POINT('Ctrl Pts',(21.1259933653335,14.3132344332075,-6.17219216889758));
#65513=CARTESIAN_POINT('Ctrl Pts',(21.1189824148079,14.3339500177816,-6.29589130954337));
#65514=CARTESIAN_POINT('Ctrl Pts',(21.1119707905225,14.3546675931453,-6.41960233780791));
#65515=CARTESIAN_POINT('Ctrl Pts',(21.104959166237,14.3699189367607,-6.54421729408242));
#65516=CARTESIAN_POINT('Ctrl Pts',(21.0979475419516,14.3796478851492,-6.66922522109208));
#65517=CARTESIAN_POINT('Ctrl Pts',(21.0909338264986,14.3893797351281,-6.79427043083558));
#65518=CARTESIAN_POINT('Ctrl Pts',(21.0839201110456,14.3935858804475,-6.91970845912758));
#65519=CARTESIAN_POINT('Ctrl Pts',(21.0769063955927,14.3922622147059,-7.04502555802502));
#65520=CARTESIAN_POINT('Ctrl Pts',(21.069804034079,14.3909218192076,-7.17192653457186));
#65521=CARTESIAN_POINT('Ctrl Pts',(21.0627016725654,14.3839108701113,-7.29870309586766));
#65522=CARTESIAN_POINT('Ctrl Pts',(21.0555993110518,14.37127938786,-7.42482540499111));
#65523=CARTESIAN_POINT('Ctrl Pts',(21.0485733953341,14.358783863728,-7.54959020502676));
#65524=CARTESIAN_POINT('Ctrl Pts',(21.0415474796164,14.3407883237577,-7.67371439178308));
#65525=CARTESIAN_POINT('Ctrl Pts',(21.0345215638987,14.3173929110686,-7.79669439901484));
#65526=CARTESIAN_POINT('Ctrl Pts',(21.0273809794871,14.2936156660999,-7.92168154059925));
#65527=CARTESIAN_POINT('Ctrl Pts',(21.0202403950756,14.264260841247,-8.04548642037499));
#65528=CARTESIAN_POINT('Ctrl Pts',(21.013099810664,14.2294863484673,-8.16759622403539));
#65529=CARTESIAN_POINT('Ctrl Pts',(21.0059592262525,14.1947118556876,-8.28970602769578));
#65530=CARTESIAN_POINT('Ctrl Pts',(20.9988186418409,14.1545178775712,-8.41012037987649));
#65531=CARTESIAN_POINT('Ctrl Pts',(20.9916780574294,14.1091131539846,-8.52834817519842));
#65532=CARTESIAN_POINT('Ctrl Pts',(20.9848875792511,14.0659346454851,-8.64077920575989));
#65533=CARTESIAN_POINT('Ctrl Pts',(20.9780971010728,14.0179001275206,-8.75160660314064));
#65534=CARTESIAN_POINT('Ctrl Pts',(20.9713066228945,13.9651477064359,-8.86036976757665));
#65535=CARTESIAN_POINT('Ctrl Pts',(20.9645253559579,13.9124668436842,-8.96898539545253));
#65536=CARTESIAN_POINT('Ctrl Pts',(20.9577440890213,13.8550809778343,-9.07554198259683));
#65537=CARTESIAN_POINT('Ctrl Pts',(20.9509628220846,13.793177528671,-9.17959536747338));
#65538=CARTESIAN_POINT('Ctrl Pts',(20.9441888767195,13.7313409151793,-9.28353640840212));
#65539=CARTESIAN_POINT('Ctrl Pts',(20.9374149313544,13.6649966269885,-9.38497926183249));
#65540=CARTESIAN_POINT('Ctrl Pts',(20.9306409859893,13.5943792727532,-9.48350168617723));
#65541=CARTESIAN_POINT('Ctrl Pts',(20.9238724821202,13.5238186452894,-9.58194496766671));
#65542=CARTESIAN_POINT('Ctrl Pts',(20.9171039782511,13.4489920202032,-9.67747214528359));
#65543=CARTESIAN_POINT('Ctrl Pts',(20.910335474382,13.370178451617,-9.76968810035086));
#65544=CARTESIAN_POINT('Ctrl Pts',(20.903569799622,13.2913978256411,-9.8618655108588));
#65545=CARTESIAN_POINT('Ctrl Pts',(20.896804124862,13.2086338378673,-9.95073412927473));
#65546=CARTESIAN_POINT('Ctrl Pts',(20.890038450102,13.1222067694605,-10.0359306961828));
#65547=CARTESIAN_POINT('Ctrl Pts',(20.8832740089491,13.035795459577,-10.1211117289289));
#65548=CARTESIAN_POINT('Ctrl Pts',(20.8765095677961,12.9457226947661,-10.2026217459866));
#65549=CARTESIAN_POINT('Ctrl Pts',(20.8697451266432,12.8523461041995,-10.2801338528855));
#65550=CARTESIAN_POINT('Ctrl Pts',(20.8629802282965,12.7589632025141,-10.3576511986577));
#65551=CARTESIAN_POINT('Ctrl Pts',(20.8562153299499,12.6622763543278,-10.4311698294127));
#65552=CARTESIAN_POINT('Ctrl Pts',(20.8494504316032,12.5626761707932,-10.5004032227565));
#65553=CARTESIAN_POINT('Ctrl Pts',(20.8426833849945,12.4630443582094,-10.5696586018671));
#65554=CARTESIAN_POINT('Ctrl Pts',(20.8359163383857,12.3604977161624,-10.6346258000381));
#65555=CARTESIAN_POINT('Ctrl Pts',(20.8291492917769,12.2554550341066,-10.6950621365488));
#65556=CARTESIAN_POINT('Ctrl Pts',(20.8223742557459,12.1502883348272,-10.7555698264038));
#65557=CARTESIAN_POINT('Ctrl Pts',(20.815599219715,12.0426200781834,-10.8115357695555));
#65558=CARTESIAN_POINT('Ctrl Pts',(20.808824183684,11.9328928762342,-10.8627636652982));
#65559=CARTESIAN_POINT('Ctrl Pts',(20.8020445915196,11.8230918840095,-10.9140260112088));
#65560=CARTESIAN_POINT('Ctrl Pts',(20.7952649993552,11.7112295779413,-10.9605438102634));
#65561=CARTESIAN_POINT('Ctrl Pts',(20.7884854071908,11.5977659401151,-11.002169927564));
#65562=CARTESIAN_POINT('Ctrl Pts',(20.7816949968921,11.4841212493811,-11.0438624672861));
#65563=CARTESIAN_POINT('Ctrl Pts',(20.7749045865934,11.3688705257193,-11.0806476224473));
#65564=CARTESIAN_POINT('Ctrl Pts',(20.7681141762946,11.2524863546908,-11.1124288014722));
#65565=CARTESIAN_POINT('Ctrl Pts',(20.7650717067341,11.2003399773581,-11.1266684814808));
#65566=CARTESIAN_POINT('Ctrl Pts',(20.7620292371736,11.1479661589978,-11.1399042936374));
#65567=CARTESIAN_POINT('Ctrl Pts',(20.7589867676131,11.0954077443162,-11.1521309263401));
#65568=CARTESIAN_POINT('Ctrl Pts',(20.7486384526106,10.9166414426865,-11.193717224612));
#65569=CARTESIAN_POINT('Ctrl Pts',(20.7382901376082,10.7352286283145,-11.223745455636));
#65570=CARTESIAN_POINT('Ctrl Pts',(20.7279418226057,10.5523855434177,-11.2419732221183));
#65571=CARTESIAN_POINT('Ctrl Pts',(20.7200673248741,10.4132520268103,-11.2558435484257));
#65572=CARTESIAN_POINT('Ctrl Pts',(20.7121928271425,10.2732902767665,-11.2628818332749));
#65573=CARTESIAN_POINT('Ctrl Pts',(20.7043183294109,10.1330470789259,-11.2629985243055));
#65574=CARTESIAN_POINT('Ctrl Pts',(20.7043183293681,10.1330470781642,-11.2629985243062));
#65575=CARTESIAN_POINT('Ctrl Pts',(20.6972124859225,10.0064934563144,-11.2631038247387));
#65576=CARTESIAN_POINT('Ctrl Pts',(20.6901066424768,9.87976518847473,-11.2575689158587));
#65577=CARTESIAN_POINT('Ctrl Pts',(20.6830007990312,9.75340734194371,-11.2463776695622));
#65578=CARTESIAN_POINT('Ctrl Pts',(20.6761360072116,9.63133593439973,-11.2355660640696));
#65579=CARTESIAN_POINT('Ctrl Pts',(20.6692712153921,9.50961067676056,-11.2194756600415));
#65580=CARTESIAN_POINT('Ctrl Pts',(20.6624064235726,9.38872389838046,-11.1981448006553));
#65581=CARTESIAN_POINT('Ctrl Pts',(20.6555457687443,9.26790997108627,-11.1768267960766));
#65582=CARTESIAN_POINT('Ctrl Pts',(20.6486851139159,9.14793391910229,-11.1502746878193));
#65583=CARTESIAN_POINT('Ctrl Pts',(20.6418244590876,9.0292818698926,-11.1185785249504));
#65584=CARTESIAN_POINT('Ctrl Pts',(20.6349664011617,8.9106747329837,-11.0868943597471));
#65585=CARTESIAN_POINT('Ctrl Pts',(20.6281083432358,8.79339099550801,-11.0500701203385));
#65586=CARTESIAN_POINT('Ctrl Pts',(20.6212502853099,8.67790488099607,-11.0082465755594));
#65587=CARTESIAN_POINT('Ctrl Pts',(20.6205162595467,8.66554427041757,-11.003770153851));
#65588=CARTESIAN_POINT('Ctrl Pts',(20.6197822337835,8.65320423875188,-10.9992365089288));
#65589=CARTESIAN_POINT('Ctrl Pts',(20.6190482080202,8.64088535679775,-10.9946458471364));
#65590=CARTESIAN_POINT('Origin',(23.734,10.1295,-7.));
#65591=CARTESIAN_POINT('',(19.1191572628085,8.64088535679774,-10.9946458471364));
#65592=CARTESIAN_POINT('',(19.5287462306467,8.64088535560039,-10.9946458466902));
#65593=CARTESIAN_POINT('',(23.734,8.64088535679774,-10.9946458471364));
#65594=CARTESIAN_POINT('',(19.613681670589,10.1293184243372,-11.262999996133));
#65595=CARTESIAN_POINT('Ctrl Pts',(19.5287462306467,8.64088535560039,-10.9946458466902));
#65596=CARTESIAN_POINT('Ctrl Pts',(19.5427562929707,8.87611781401766,-11.0823058035117));
#65597=CARTESIAN_POINT('Ctrl Pts',(19.5565690978808,9.11863897266564,-11.1490184691121));
#65598=CARTESIAN_POINT('Ctrl Pts',(19.5847929390305,9.61761196897248,-11.2398990512266));
#65599=CARTESIAN_POINT('Ctrl Pts',(19.5992904570035,9.873209923916,-11.2629888770781));
#65600=CARTESIAN_POINT('Ctrl Pts',(19.6137437552536,10.1293149200936,-11.2629999959823));
#65601=CARTESIAN_POINT('Ctrl Pts',(19.613681670589,10.1293184243372,-11.262999996133));
#65602=CARTESIAN_POINT('Ctrl Pts',(19.6210623037642,10.2610687195736,-11.263005607826));
#65603=CARTESIAN_POINT('Ctrl Pts',(19.6284429369393,10.3928267771473,-11.2568991564636));
#65604=CARTESIAN_POINT('Ctrl Pts',(19.6358235701145,10.5240278125494,-11.2447045604052));
#65605=CARTESIAN_POINT('Ctrl Pts',(19.6432028342893,10.6552045120622,-11.2325122262675));
#65606=CARTESIAN_POINT('Ctrl Pts',(19.650582098464,10.7858240783452,-11.2142340323102));
#65607=CARTESIAN_POINT('Ctrl Pts',(19.6579613626388,10.9153264213143,-11.1899458034161));
#65608=CARTESIAN_POINT('Ctrl Pts',(19.6653396985726,11.044812474126,-11.1656606297492));
#65609=CARTESIAN_POINT('Ctrl Pts',(19.6727180345064,11.1731812706445,-11.1353669878975));
#65610=CARTESIAN_POINT('Ctrl Pts',(19.6800963704403,11.2998820511657,-11.0991919757812));
#65611=CARTESIAN_POINT('Ctrl Pts',(19.6849288196367,11.382864866059,-11.0754991119973));
#65612=CARTESIAN_POINT('Ctrl Pts',(19.6897612688331,11.4651323638681,-11.0492844183613));
#65613=CARTESIAN_POINT('Ctrl Pts',(19.6945937180296,11.5465329042847,-11.0205953226076));
#65614=CARTESIAN_POINT('Ctrl Pts',(19.7016231773756,11.6649411412557,-10.9788631027588));
#65615=CARTESIAN_POINT('Ctrl Pts',(19.7086526367216,11.7815525661295,-10.9318790465684));
#65616=CARTESIAN_POINT('Ctrl Pts',(19.7156820960676,11.8958854944383,-10.8798261926326));
#65617=CARTESIAN_POINT('Ctrl Pts',(19.722709782053,12.0101895793458,-10.8277864703587));
#65618=CARTESIAN_POINT('Ctrl Pts',(19.7297374680383,12.1222159630139,-10.7706806571767));
#65619=CARTESIAN_POINT('Ctrl Pts',(19.7367651540237,12.2315037832726,-10.7087395561171));
#65620=CARTESIAN_POINT('Ctrl Pts',(19.7437942650805,12.3408137648732,-10.6467858946649));
#65621=CARTESIAN_POINT('Ctrl Pts',(19.7508233761373,12.4473837362772,-10.5799951717423));
#65622=CARTESIAN_POINT('Ctrl Pts',(19.7578524871941,12.5507782076321,-10.5086437324479));
#65623=CARTESIAN_POINT('Ctrl Pts',(19.7648822673835,12.6541825215712,-10.4372855008895));
#65624=CARTESIAN_POINT('Ctrl Pts',(19.771912047573,12.7544104201016,-10.3613659117439));
#65625=CARTESIAN_POINT('Ctrl Pts',(19.7789418277624,12.8510567997471,-10.2812036794065));
#65626=CARTESIAN_POINT('Ctrl Pts',(19.7859761861195,12.947766120667,-10.20098924115));
#65627=CARTESIAN_POINT('Ctrl Pts',(19.7930105444766,13.0408889712832,-10.116526891086));
#65628=CARTESIAN_POINT('Ctrl Pts',(19.8000449028336,13.1300544842105,-10.0281746626118));
#65629=CARTESIAN_POINT('Ctrl Pts',(19.803676389535,13.176086170113,-9.9825628347157));
#65630=CARTESIAN_POINT('Ctrl Pts',(19.8073078762364,13.2210637677684,-9.93591490652767));
#65631=CARTESIAN_POINT('Ctrl Pts',(19.8109393629378,13.2649402640227,-9.88828380716734));
#65632=CARTESIAN_POINT('Ctrl Pts',(19.8185510511639,13.3569065129464,-9.788447814911));
#65633=CARTESIAN_POINT('Ctrl Pts',(19.82616273939,13.4440921851538,-9.68422623732347));
#65634=CARTESIAN_POINT('Ctrl Pts',(19.8337744276161,13.5261126987745,-9.57608058385672));
#65635=CARTESIAN_POINT('Ctrl Pts',(19.8415669759686,13.6100820889147,-9.46536529853304));
#65636=CARTESIAN_POINT('Ctrl Pts',(19.8493595243211,13.6886375971267,-9.350537337596));
#65637=CARTESIAN_POINT('Ctrl Pts',(19.8571520726736,13.7614114960694,-9.23212631468719));
#65638=CARTESIAN_POINT('Ctrl Pts',(19.8647577752929,13.8324404597364,-9.11655449063818));
#65639=CARTESIAN_POINT('Ctrl Pts',(19.8723634779121,13.8979617722854,-8.99756971412403));
#65640=CARTESIAN_POINT('Ctrl Pts',(19.8799691805314,13.9576776738065,-8.87569312462606));
#65641=CARTESIAN_POINT('Ctrl Pts',(19.8878551517505,14.0195940941942,-8.74932540750959));
#65642=CARTESIAN_POINT('Ctrl Pts',(19.8957411229696,14.0752688994055,-8.61984891580091));
#65643=CARTESIAN_POINT('Ctrl Pts',(19.9036270941887,14.1244221857155,-8.48787288774221));
#65644=CARTESIAN_POINT('Ctrl Pts',(19.9115130654078,14.1735754720254,-8.35589685968352));
#65645=CARTESIAN_POINT('Ctrl Pts',(19.9193990366269,14.2162070893851,-8.22142157961869));
#65646=CARTESIAN_POINT('Ctrl Pts',(19.9272850078459,14.2520924147731,-8.08508100234748));
#65647=CARTESIAN_POINT('Ctrl Pts',(19.9343239536661,14.2841233281666,-7.9633846494403));
#65648=CARTESIAN_POINT('Ctrl Pts',(19.9413628994862,14.3107676181272,-7.8402454199408));
#65649=CARTESIAN_POINT('Ctrl Pts',(19.9484018453063,14.3319126474473,-7.71616823482706));
#65650=CARTESIAN_POINT('Ctrl Pts',(19.9554405817332,14.3530570477492,-7.59209474073655));
#65651=CARTESIAN_POINT('Ctrl Pts',(19.9624793181602,14.3687024503286,-7.4670837237731));
#65652=CARTESIAN_POINT('Ctrl Pts',(19.9695180545871,14.3787875954937,-7.34164884133137));
#65653=CARTESIAN_POINT('Ctrl Pts',(19.976560483799,14.3888780317039,-7.21614815104951));
#65654=CARTESIAN_POINT('Ctrl Pts',(19.9836029130109,14.3934023507515,-7.09022353254098));
#65655=CARTESIAN_POINT('Ctrl Pts',(19.9906453422228,14.3923512886368,-6.96439254336727));
#65656=CARTESIAN_POINT('Ctrl Pts',(19.9976897288499,14.3912999343835,-6.83852657996872));
#65657=CARTESIAN_POINT('Ctrl Pts',(20.0047341154771,14.384670122848,-6.71275468020004));
#65658=CARTESIAN_POINT('Ctrl Pts',(20.0117785021043,14.3725046893258,-6.58759218441076));
#65659=CARTESIAN_POINT('Ctrl Pts',(20.0188293217025,14.3603281462655,-6.46231538956881));
#65660=CARTESIAN_POINT('Ctrl Pts',(20.0258801413008,14.3426059296771,-6.33764949029167));
#65661=CARTESIAN_POINT('Ctrl Pts',(20.032930960899,14.3194325420246,-6.21410287360031));
#65662=CARTESIAN_POINT('Ctrl Pts',(20.0364975248507,14.3077105900036,-6.15160844961165));
#65663=CARTESIAN_POINT('Ctrl Pts',(20.0400640888024,14.2945946542908,-6.08940024916908));
#65664=CARTESIAN_POINT('Ctrl Pts',(20.043630652754,14.2801018815878,-6.02754279242752));
#65665=CARTESIAN_POINT('Ctrl Pts',(20.0506540757907,14.2515621231407,-5.9057305685185));
#65666=CARTESIAN_POINT('Ctrl Pts',(20.0576774988273,14.2176287610004,-5.78506067889005));
#65667=CARTESIAN_POINT('Ctrl Pts',(20.064700921864,14.178413687597,-5.66603337733305));
#65668=CARTESIAN_POINT('Ctrl Pts',(20.0717185186296,14.1392311450044,-5.54710481471211));
#65669=CARTESIAN_POINT('Ctrl Pts',(20.0787361153952,14.0947757355895,-5.42981649293811));
#65670=CARTESIAN_POINT('Ctrl Pts',(20.0857537121608,14.0452096568303,-5.31465526274116));
#65671=CARTESIAN_POINT('Ctrl Pts',(20.0927670515899,13.9956736481201,-5.19956389693379));
#65672=CARTESIAN_POINT('Ctrl Pts',(20.0997803910189,13.9410332971071,-5.08659740716836));
#65673=CARTESIAN_POINT('Ctrl Pts',(20.106793730448,13.8814994526977,-4.97622404724333));
#65674=CARTESIAN_POINT('Ctrl Pts',(20.1138574059531,13.821538322521,-4.86505851664211));
#65675=CARTESIAN_POINT('Ctrl Pts',(20.1209210814582,13.7566133174844,-4.75652385852162));
#65676=CARTESIAN_POINT('Ctrl Pts',(20.1279847569633,13.6869877988477,-4.65107480726828));
#65677=CARTESIAN_POINT('Ctrl Pts',(20.1349957098057,13.6178819590572,-4.54641281860872));
#65678=CARTESIAN_POINT('Ctrl Pts',(20.1420066626481,13.5441457768754,-4.4447908421696));
#65679=CARTESIAN_POINT('Ctrl Pts',(20.1490176154904,13.4660808058284,-4.34662525711552));
#65680=CARTESIAN_POINT('Ctrl Pts',(20.1560292419106,13.3880083346838,-4.24845024079589));
#65681=CARTESIAN_POINT('Ctrl Pts',(20.1630408683308,13.3056064871499,-4.15373257998509));
#65682=CARTESIAN_POINT('Ctrl Pts',(20.1700524947509,13.2192173973556,-4.06285591016064));
#65683=CARTESIAN_POINT('Ctrl Pts',(20.1770662121528,13.1328025449214,-3.97195213942652));
#65684=CARTESIAN_POINT('Ctrl Pts',(20.1840799295547,13.0423983490892,-3.8848919206958));
#65685=CARTESIAN_POINT('Ctrl Pts',(20.1910936469566,12.9483838509154,-3.80202207089415));
#65686=CARTESIAN_POINT('Ctrl Pts',(20.1981960049244,12.8531811813556,-3.71810489768801));
#65687=CARTESIAN_POINT('Ctrl Pts',(20.2052983628922,12.7542766304511,-3.63848501133126));
#65688=CARTESIAN_POINT('Ctrl Pts',(20.2124007208601,12.6520974127302,-3.56347976969624));
#65689=CARTESIAN_POINT('Ctrl Pts',(20.2194266380452,12.5510179226514,-3.48928178945322));
#65690=CARTESIAN_POINT('Ctrl Pts',(20.2264525552303,12.4467342673697,-3.41959977243168));
#65691=CARTESIAN_POINT('Ctrl Pts',(20.2334784724154,12.3396876781542,-3.35469625033312));
#65692=CARTESIAN_POINT('Ctrl Pts',(20.2406190507746,12.2308941159415,-3.28873351932974));
#65693=CARTESIAN_POINT('Ctrl Pts',(20.2477596291338,12.1192470170137,-3.22770681705742));
#65694=CARTESIAN_POINT('Ctrl Pts',(20.254900207493,12.0052331387805,-3.17184193219762));
#65695=CARTESIAN_POINT('Ctrl Pts',(20.2620407858522,11.8912192605474,-3.11597704733782));
#65696=CARTESIAN_POINT('Ctrl Pts',(20.2691813642114,11.7748390041325,-3.06527409536859));
#65697=CARTESIAN_POINT('Ctrl Pts',(20.2763219425706,11.6565970046819,-3.01990656663797));
#65698=CARTESIAN_POINT('Ctrl Pts',(20.2831124368812,11.5441521039813,-2.97676329024846));
#65699=CARTESIAN_POINT('Ctrl Pts',(20.2899029311918,11.4296496272437,-2.93830180029273));
#65700=CARTESIAN_POINT('Ctrl Pts',(20.2966934255024,11.3135242806343,-2.90472766438319));
#65701=CARTESIAN_POINT('Ctrl Pts',(20.3034747086535,11.1975564555602,-2.87119907106695));
#65702=CARTESIAN_POINT('Ctrl Pts',(20.3102559918046,11.0799705337984,-2.84254477101641));
#65703=CARTESIAN_POINT('Ctrl Pts',(20.3170372749558,10.9612220024664,-2.81892268540592));
#65704=CARTESIAN_POINT('Ctrl Pts',(20.3238112366047,10.8426016795597,-2.79532610369315));
#65705=CARTESIAN_POINT('Ctrl Pts',(20.3305851982536,10.7228216505048,-2.77675101741854));
#65706=CARTESIAN_POINT('Ctrl Pts',(20.3373591599025,10.602352688061,-2.76330561222627));
#65707=CARTESIAN_POINT('Ctrl Pts',(20.3441276801126,10.48198049683,-2.74987100756003));
#65708=CARTESIAN_POINT('Ctrl Pts',(20.3508962003228,10.3609208876254,-2.74155793704571));
#65709=CARTESIAN_POINT('Ctrl Pts',(20.3576647205329,10.2396542166227,-2.73842340810819));
#65710=CARTESIAN_POINT('Ctrl Pts',(20.3644304116747,10.1184382319863,-2.73529018932358));
#65711=CARTESIAN_POINT('Ctrl Pts',(20.3711961028166,9.99701577598613,-2.73733122414958));
#65712=CARTESIAN_POINT('Ctrl Pts',(20.3779617939584,9.8758711148973,-2.74455156433055));
#65713=CARTESIAN_POINT('Ctrl Pts',(20.3847262515225,9.7547485419237,-2.75177058803827));
#65714=CARTESIAN_POINT('Ctrl Pts',(20.3914907090865,9.63390408190446,-2.76416701590755));
#65715=CARTESIAN_POINT('Ctrl Pts',(20.3982551666505,9.51381996728511,-2.78169381181069));
#65716=CARTESIAN_POINT('Ctrl Pts',(20.4050200814275,9.39372773612192,-2.79922179235852));
#65717=CARTESIAN_POINT('Ctrl Pts',(20.4117849962045,9.27439636769387,-2.82188076925702));
#65718=CARTESIAN_POINT('Ctrl Pts',(20.4185499109815,9.15630016132667,-2.8495721818099));
#65719=CARTESIAN_POINT('Ctrl Pts',(20.4253169740298,9.03816645224213,-2.87727238806794));
#65720=CARTESIAN_POINT('Ctrl Pts',(20.4320840370781,8.92126909293508,-2.91000810994903));
#65721=CARTESIAN_POINT('Ctrl Pts',(20.4388511001264,8.8060686569394,-2.94763051040446));
#65722=CARTESIAN_POINT('Ctrl Pts',(20.4456261525318,8.69073221254255,-2.98529732876934));
#65723=CARTESIAN_POINT('Ctrl Pts',(20.4524012049372,8.57709708877692,-3.02786220934678));
#65724=CARTESIAN_POINT('Ctrl Pts',(20.4591762573426,8.46560533251585,-3.07512757716664));
#65725=CARTESIAN_POINT('Ctrl Pts',(20.465955865875,8.3540385996251,-3.12242473027806));
#65726=CARTESIAN_POINT('Ctrl Pts',(20.4727354744074,8.24461847941592,-3.17442847978152));
#65727=CARTESIAN_POINT('Ctrl Pts',(20.4795150829397,8.13776210427539,-3.23089544391052));
#65728=CARTESIAN_POINT('Ctrl Pts',(20.4863055094517,8.03073522222619,-3.28745251036128));
#65729=CARTESIAN_POINT('Ctrl Pts',(20.4930959359638,7.92628060892515,-3.34848679214083));
#65730=CARTESIAN_POINT('Ctrl Pts',(20.4998863624758,7.82478626913523,-3.41371172118535));
#65731=CARTESIAN_POINT('Ctrl Pts',(20.5029286524462,7.77931413105292,-3.44293420774036));
#65732=CARTESIAN_POINT('Ctrl Pts',(20.5059709424165,7.73443575525086,-3.4729973349816));
#65733=CARTESIAN_POINT('Ctrl Pts',(20.5090132323869,7.69018375192213,-3.50387282241288));
#65734=CARTESIAN_POINT('Ctrl Pts',(20.5160528480572,7.58778815547792,-3.57531623091908));
#65735=CARTESIAN_POINT('Ctrl Pts',(20.5230924637274,7.48839576824068,-3.65135791091549));
#65736=CARTESIAN_POINT('Ctrl Pts',(20.5301320793977,7.39243615095284,-3.73172056178803));
#65737=CARTESIAN_POINT('Ctrl Pts',(20.5371627089137,7.29659902727188,-3.81198062876912));
#65738=CARTESIAN_POINT('Ctrl Pts',(20.5441933384298,7.20418624476916,-3.89655044007299));
#65739=CARTESIAN_POINT('Ctrl Pts',(20.5512239679459,7.11559764941311,-3.98511001508732));
#65740=CARTESIAN_POINT('Ctrl Pts',(20.5582471924636,7.0271023598425,-4.07357631488181));
#65741=CARTESIAN_POINT('Ctrl Pts',(20.5652704169812,6.94242351009667,-4.16602373977542));
#65742=CARTESIAN_POINT('Ctrl Pts',(20.5722936414989,6.86192690158119,-4.26209294414699));
#65743=CARTESIAN_POINT('Ctrl Pts',(20.5793524281949,6.78102269755993,-4.3586485960431));
#65744=CARTESIAN_POINT('Ctrl Pts',(20.5864112148909,6.70434351288937,-4.45886255685475));
#65745=CARTESIAN_POINT('Ctrl Pts',(20.5934700015869,6.63222286897191,-4.56233274034623));
#65746=CARTESIAN_POINT('Ctrl Pts',(20.6004830794517,6.56056923879038,-4.66513290767694));
#65747=CARTESIAN_POINT('Ctrl Pts',(20.6074961573164,6.49341550627245,-4.77114692695205));
#65748=CARTESIAN_POINT('Ctrl Pts',(20.6145092351811,6.4310476922353,-4.87994822535157));
#65749=CARTESIAN_POINT('Ctrl Pts',(20.6215200654578,6.36869986616283,-4.9887146545394));
#65750=CARTESIAN_POINT('Ctrl Pts',(20.6285308957345,6.31113509680343,-5.10026624921301));
#65751=CARTESIAN_POINT('Ctrl Pts',(20.6355417260111,6.25859484105923,-5.21414943220723));
#65752=CARTESIAN_POINT('Ctrl Pts',(20.6425517265455,6.20606080353314,-5.32801913695587));
#65753=CARTESIAN_POINT('Ctrl Pts',(20.6495617270799,6.15855025661158,-5.44421952922821));
#65754=CARTESIAN_POINT('Ctrl Pts',(20.6565717276143,6.11625749444774,-5.56227485532575));
#65755=CARTESIAN_POINT('Ctrl Pts',(20.6636661271634,6.07345553582416,-5.68175154411103));
#65756=CARTESIAN_POINT('Ctrl Pts',(20.6707605267125,6.0359979916284,-5.80312775504321));
#65757=CARTESIAN_POINT('Ctrl Pts',(20.6778549262616,6.00403488298935,-5.92589266442861));
#65758=CARTESIAN_POINT('Ctrl Pts',(20.6848699695753,5.97242930594331,-6.04728435526654));
#65759=CARTESIAN_POINT('Ctrl Pts',(20.691885012889,5.94619591700699,-6.17003344375839));
#65760=CARTESIAN_POINT('Ctrl Pts',(20.6989000562027,5.92542852701159,-6.29363462004067));
#65761=CARTESIAN_POINT('Ctrl Pts',(20.7060341338695,5.90430874677111,-6.41933311566898));
#65762=CARTESIAN_POINT('Ctrl Pts',(20.7131682115363,5.88884222559255,-6.54591246948119));
#65763=CARTESIAN_POINT('Ctrl Pts',(20.720302289203,5.87907269796409,-6.67283528596788));
#65764=CARTESIAN_POINT('Ctrl Pts',(20.7274363668698,5.86930317033562,-6.79975810245456));
#65765=CARTESIAN_POINT('Ctrl Pts',(20.7345704445365,5.86523062067719,-6.92702396271638));
#65766=CARTESIAN_POINT('Ctrl Pts',(20.7417045222033,5.86684324052786,-7.05409575700999));
#65767=CARTESIAN_POINT('Ctrl Pts',(20.7487555408127,5.86843708532577,-7.17968810799774));
#65768=CARTESIAN_POINT('Ctrl Pts',(20.7558065594222,5.87558719238043,-7.30531726205016));
#65769=CARTESIAN_POINT('Ctrl Pts',(20.7628575780316,5.88828942330491,-7.43046700701646));
#65770=CARTESIAN_POINT('Ctrl Pts',(20.7699032665315,5.90098205217249,-7.55552214695005));
#65771=CARTESIAN_POINT('Ctrl Pts',(20.7769489550314,5.91921840902034,-7.68009822009394));
#65772=CARTESIAN_POINT('Ctrl Pts',(20.7839946435314,5.94294234854903,-7.80368154829967));
#65773=CARTESIAN_POINT('Ctrl Pts',(20.7910363483395,5.96665287436202,-7.92719500144824));
#65774=CARTESIAN_POINT('Ctrl Pts',(20.7980780531477,5.99584473055009,-8.04971645279611));
#65775=CARTESIAN_POINT('Ctrl Pts',(20.8051197579558,6.03041028946687,-8.17074016972232));
#65776=CARTESIAN_POINT('Ctrl Pts',(20.8121590390629,6.06496395118215,-8.29172223120907));
#65777=CARTESIAN_POINT('Ctrl Pts',(20.81919832017,6.10488752575289,-8.41120721791972));
#65778=CARTESIAN_POINT('Ctrl Pts',(20.8262376012772,6.15002298728712,-8.528702621601));
#65779=CARTESIAN_POINT('Ctrl Pts',(20.8332767281295,6.19515745974894,-8.64619545055594));
#65780=CARTESIAN_POINT('Ctrl Pts',(20.8403158549819,6.24550345864841,-8.76169842478665));
#65781=CARTESIAN_POINT('Ctrl Pts',(20.8473549818343,6.30085412572507,-8.87473725342982));
#65782=CARTESIAN_POINT('Ctrl Pts',(20.8509200435934,6.32888722566361,-8.93198730925843));
#65783=CARTESIAN_POINT('Ctrl Pts',(20.8544851053524,6.35820328570989,-8.98860562121714));
#65784=CARTESIAN_POINT('Ctrl Pts',(20.8580501671115,6.38877083910759,-9.04453279378179));
#65785=CARTESIAN_POINT('Ctrl Pts',(20.8656419313286,6.45386414569605,-9.16362916184931));
#65786=CARTESIAN_POINT('Ctrl Pts',(20.8732336955456,6.52461037034494,-9.27954435589301));
#65787=CARTESIAN_POINT('Ctrl Pts',(20.8808254597627,6.60067979658225,-9.39177694862015));
#65788=CARTESIAN_POINT('Ctrl Pts',(20.8886229891175,6.67881098811066,-9.50705146338692));
#65789=CARTESIAN_POINT('Ctrl Pts',(20.8964205184722,6.7625578532525,-9.61844067454016));
#65790=CARTESIAN_POINT('Ctrl Pts',(20.904218047827,6.85151803388108,-9.72543633750618));
#65791=CARTESIAN_POINT('Ctrl Pts',(20.9118262952094,6.93831874095385,-9.82983472264376));
#65792=CARTESIAN_POINT('Ctrl Pts',(20.9194345425919,7.03008237539708,-9.93005022576152));
#65793=CARTESIAN_POINT('Ctrl Pts',(20.9270427899744,7.12639604911989,-10.0256463210706));
#65794=CARTESIAN_POINT('Ctrl Pts',(20.9349349603153,7.22630393604349,-10.1248098511419));
#65795=CARTESIAN_POINT('Ctrl Pts',(20.9428271306562,7.3311078117208,-10.219002308715));
#65796=CARTESIAN_POINT('Ctrl Pts',(20.950719300997,7.4403062336633,-10.3077796007437));
#65797=CARTESIAN_POINT('Ctrl Pts',(20.9586114713379,7.5495046556058,-10.3965568927723));
#65798=CARTESIAN_POINT('Ctrl Pts',(20.9665036416788,7.66309737480791,-10.4799188219024));
#65799=CARTESIAN_POINT('Ctrl Pts',(20.9743958120197,7.78054523318155,-10.5574682716));
#65800=CARTESIAN_POINT('Ctrl Pts',(20.9814303456134,7.88523011320223,-10.6265904756971));
#65801=CARTESIAN_POINT('Ctrl Pts',(20.9884648792071,7.99304022283171,-10.6911356375115));
#65802=CARTESIAN_POINT('Ctrl Pts',(20.9954994128008,8.10354413328733,-10.75082281988));
#65803=CARTESIAN_POINT('Ctrl Pts',(21.0025299902701,8.213985897873,-10.8104764350032));
#65804=CARTESIAN_POINT('Ctrl Pts',(21.0095605677395,8.32711810832358,-10.8652773293347));
#65805=CARTESIAN_POINT('Ctrl Pts',(21.0165911452088,8.4424828530154,-10.9149894183484));
#65806=CARTESIAN_POINT('Ctrl Pts',(21.020579512978,8.50792797917055,-10.9431905290571));
#65807=CARTESIAN_POINT('Ctrl Pts',(21.0245678807472,8.5740911029662,-10.9697548034393));
#65808=CARTESIAN_POINT('Ctrl Pts',(21.0285562485163,8.64088535679774,-10.9946458471364));
#65809=CARTESIAN_POINT('',(19.2043183294647,10.1295728822702,-11.262999999377));
#65810=CARTESIAN_POINT('Ctrl Pts',(20.6190482080202,8.64088535679775,-10.9946458471364));
#65811=CARTESIAN_POINT('Ctrl Pts',(20.6121906086773,8.52579681219007,-10.9517578166766));
#65812=CARTESIAN_POINT('Ctrl Pts',(20.6053330093343,8.412555906166,-10.9038893145581));
#65813=CARTESIAN_POINT('Ctrl Pts',(20.5984754099914,8.30161734079923,-10.8512353841583));
#65814=CARTESIAN_POINT('Ctrl Pts',(20.5916140006898,8.19061713996373,-10.7985522001832));
#65815=CARTESIAN_POINT('Ctrl Pts',(20.5847525913881,8.0819222045518,-10.7410784518095));
#65816=CARTESIAN_POINT('Ctrl Pts',(20.5778911820865,7.97596448314815,-10.6790560987375));
#65817=CARTESIAN_POINT('Ctrl Pts',(20.5710276626094,7.869974175234,-10.6170146711514));
#65818=CARTESIAN_POINT('Ctrl Pts',(20.5641641431323,7.76672310363603,-10.5504220702988));
#65819=CARTESIAN_POINT('Ctrl Pts',(20.5573006236552,7.66661480714346,-10.4795639851579));
#65820=CARTESIAN_POINT('Ctrl Pts',(20.5504298984386,7.56640141088351,-10.4086315088973));
#65821=CARTESIAN_POINT('Ctrl Pts',(20.5435591732221,7.46933770314235,-10.333424853554));
#65822=CARTESIAN_POINT('Ctrl Pts',(20.5366884480055,7.37579474398677,-10.2542704809227));
#65823=CARTESIAN_POINT('Ctrl Pts',(20.5332241246026,7.32862897147049,-10.2143596510014));
#65824=CARTESIAN_POINT('Ctrl Pts',(20.5297598011996,7.28235772638468,-10.1734457866596));
#65825=CARTESIAN_POINT('Ctrl Pts',(20.5262954777966,7.23702496054344,-10.1315742281033));
#65826=CARTESIAN_POINT('Ctrl Pts',(20.5192443736102,7.14475700001478,-10.0463510293761));
#65827=CARTESIAN_POINT('Ctrl Pts',(20.5121932694238,7.05617966494,-9.95697401157821));
#65828=CARTESIAN_POINT('Ctrl Pts',(20.5051421652374,6.97167381122514,-9.86379167564396));
#65829=CARTESIAN_POINT('Ctrl Pts',(20.4980963907359,6.88723183255123,-9.77067977300234));
#65830=CARTESIAN_POINT('Ctrl Pts',(20.4910506162344,6.80685546329167,-9.67376856212323));
#65831=CARTESIAN_POINT('Ctrl Pts',(20.4840048417328,6.73088887631933,-9.57344349656137));
#65832=CARTESIAN_POINT('Ctrl Pts',(20.4769630507529,6.65496523913739,-9.47317515252287));
#65833=CARTESIAN_POINT('Ctrl Pts',(20.4699212597729,6.58344664850125,-9.36949710276488));
#65834=CARTESIAN_POINT('Ctrl Pts',(20.462879468793,6.51663692385959,-9.26282774268419));
#65835=CARTESIAN_POINT('Ctrl Pts',(20.4558401014794,6.4498501940051,-9.15619509640896));
#65836=CARTESIAN_POINT('Ctrl Pts',(20.4488007341658,6.38776930400394,-9.04657351481714));
#65837=CARTESIAN_POINT('Ctrl Pts',(20.4417613668523,6.33065452248795,-8.93440999738582));
#65838=CARTESIAN_POINT('Ctrl Pts',(20.434722154203,6.27354099585986,-8.82224894433653));
#65839=CARTESIAN_POINT('Ctrl Pts',(20.4276829415537,6.22139353779856,-8.70754640545444));
#65840=CARTESIAN_POINT('Ctrl Pts',(20.4206437289045,6.17442620344216,-8.59077347972034));
#65841=CARTESIAN_POINT('Ctrl Pts',(20.4170790968991,6.15064211400004,-8.53164008950059));
#65842=CARTESIAN_POINT('Ctrl Pts',(20.4135144648938,6.12818565038781,-8.47197612678181));
#65843=CARTESIAN_POINT('Ctrl Pts',(20.4099498328884,6.10707988819629,-8.41184469548072));
#65844=CARTESIAN_POINT('Ctrl Pts',(20.4023582696467,6.06213114504391,-8.28378335202333));
#65845=CARTESIAN_POINT('Ctrl Pts',(20.3947667064051,6.02332867012886,-8.15364975670661));
#65846=CARTESIAN_POINT('Ctrl Pts',(20.3871751431634,5.99082447735158,-8.02202442154324));
#65847=CARTESIAN_POINT('Ctrl Pts',(20.3793775635648,5.95743820071792,-7.88682709848179));
#65848=CARTESIAN_POINT('Ctrl Pts',(20.3715799839662,5.93069696443189,-7.75005621879711));
#65849=CARTESIAN_POINT('Ctrl Pts',(20.3637824043676,5.91070925233697,-7.61235090220622));
#65850=CARTESIAN_POINT('Ctrl Pts',(20.3561743707007,5.89120740761466,-7.47799296824972));
#65851=CARTESIAN_POINT('Ctrl Pts',(20.3485663370339,5.8781345404609,-7.34274577259572));
#65852=CARTESIAN_POINT('Ctrl Pts',(20.340958303367,5.87153877916962,-7.20720820906679));
#65853=CARTESIAN_POINT('Ctrl Pts',(20.3330659508026,5.86469652848814,-7.06660548779349));
#65854=CARTESIAN_POINT('Ctrl Pts',(20.3251735982381,5.86482489394197,-6.92569058452576));
#65855=CARTESIAN_POINT('Ctrl Pts',(20.3172812456736,5.87191837083124,-6.78513336470115));
#65856=CARTESIAN_POINT('Ctrl Pts',(20.3093888931092,5.8790118477205,-6.64457614487654));
#65857=CARTESIAN_POINT('Ctrl Pts',(20.3014965405447,5.89307041607502,-6.50437692574409));
#65858=CARTESIAN_POINT('Ctrl Pts',(20.2936041879802,5.91402841188901,-6.36520216617491));
#65859=CARTESIAN_POINT('Ctrl Pts',(20.2865695905002,5.93270865498951,-6.24115317001707));
#65860=CARTESIAN_POINT('Ctrl Pts',(20.2795349930202,5.95688158865839,-6.11784437235239));
#65861=CARTESIAN_POINT('Ctrl Pts',(20.2725003955402,5.98646729786239,-5.99578437125368));
#65862=CARTESIAN_POINT('Ctrl Pts',(20.2654696839918,6.01603666383682,-5.87379179644538));
#65863=CARTESIAN_POINT('Ctrl Pts',(20.2584389724434,6.05101276049188,-5.75304701753563));
#65864=CARTESIAN_POINT('Ctrl Pts',(20.2514082608949,6.09126461877634,-5.63404831497107));
#65865=CARTESIAN_POINT('Ctrl Pts',(20.2443792951667,6.13150648198313,-5.5150791613845));
#65866=CARTESIAN_POINT('Ctrl Pts',(20.2373503294385,6.17702137841485,-5.39785558600509));
#65867=CARTESIAN_POINT('Ctrl Pts',(20.2303213637103,6.22762857144207,-5.28286041481675));
#65868=CARTESIAN_POINT('Ctrl Pts',(20.2232935368354,6.27822756494623,-5.167883875477));
#65869=CARTESIAN_POINT('Ctrl Pts',(20.2162657099604,6.33391705385406,-5.05513537191307));
#65870=CARTESIAN_POINT('Ctrl Pts',(20.2092378830855,6.39446848337008,-4.94507699176315));
#65871=CARTESIAN_POINT('Ctrl Pts',(20.202208203391,6.45503587669273,-4.83498959577145));
#65872=CARTESIAN_POINT('Ctrl Pts',(20.1951785236966,6.52046758537476,-4.72759407695164));
#65873=CARTESIAN_POINT('Ctrl Pts',(20.1881488440021,6.59048948921103,-4.62332719868191));
#65874=CARTESIAN_POINT('Ctrl Pts',(20.1845187436921,6.626648538538,-4.56948417260053));
#65875=CARTESIAN_POINT('Ctrl Pts',(20.1808886433821,6.66403091020618,-4.51647499565652));
#65876=CARTESIAN_POINT('Ctrl Pts',(20.177258543072,6.70259439411009,-4.46435669536894));
#65877=CARTESIAN_POINT('Ctrl Pts',(20.1698761111912,6.78101985585918,-4.35836518858973));
#65878=CARTESIAN_POINT('Ctrl Pts',(20.1624936793103,6.86435866190934,-4.25602485199227));
#65879=CARTESIAN_POINT('Ctrl Pts',(20.1551112474295,6.95225090147646,-4.15777249926552));
#65880=CARTESIAN_POINT('Ctrl Pts',(20.1477279447581,7.04015350832238,-4.05950855723876));
#65881=CARTESIAN_POINT('Ctrl Pts',(20.1403446420867,7.13261040743368,-3.96533379717853));
#65882=CARTESIAN_POINT('Ctrl Pts',(20.1329613394153,7.22922309246197,-3.87565001006583));
#65883=CARTESIAN_POINT('Ctrl Pts',(20.125576061468,7.32586162455663,-3.78594222959454));
#65884=CARTESIAN_POINT('Ctrl Pts',(20.1181907835206,7.42665793153525,-3.7007280395822));
#65885=CARTESIAN_POINT('Ctrl Pts',(20.1108055055733,7.53117808025158,-3.62037099649164));
#65886=CARTESIAN_POINT('Ctrl Pts',(20.1034200529725,7.63570070075121,-3.54001205304791));
#65887=CARTESIAN_POINT('Ctrl Pts',(20.0960346003717,7.74394708454327,-3.46451067662804));
#65888=CARTESIAN_POINT('Ctrl Pts',(20.0886491477709,7.855451839869,-3.39418886165612));
#65889=CARTESIAN_POINT('Ctrl Pts',(20.0812627355946,7.96697108276045,-3.32385790992663));
#65890=CARTESIAN_POINT('Ctrl Pts',(20.0738763234183,8.08174927371947,-3.25870803300175));
#65891=CARTESIAN_POINT('Ctrl Pts',(20.066489911242,8.19929334163063,-3.19901706712769));
#65892=CARTESIAN_POINT('Ctrl Pts',(20.0646309068826,8.22887670760733,-3.1839941083316));
#65893=CARTESIAN_POINT('Ctrl Pts',(20.0627719025232,8.25863514608028,-3.16931670369317));
#65894=CARTESIAN_POINT('Ctrl Pts',(20.0609128981638,8.28856055418469,-3.15498882227357));
#65895=CARTESIAN_POINT('Ctrl Pts',(20.0537145950365,8.40443556957037,-3.09950942917227));
#65896=CARTESIAN_POINT('Ctrl Pts',(20.0465162919091,8.52285398389169,-3.04925596260064));
#65897=CARTESIAN_POINT('Ctrl Pts',(20.0393179887818,8.6433237577775,-3.00444632409307));
#65898=CARTESIAN_POINT('Ctrl Pts',(20.032121772119,8.76375861289033,-2.95964967388574));
#65899=CARTESIAN_POINT('Ctrl Pts',(20.0249255554562,8.88624330867259,-2.92029382958354));
#65900=CARTESIAN_POINT('Ctrl Pts',(20.0177293387934,9.01026695320274,-2.88654811782648));
#65901=CARTESIAN_POINT('Ctrl Pts',(20.0105333517354,9.13428664059432,-2.85280348277102));
#65902=CARTESIAN_POINT('Ctrl Pts',(20.0033373646774,9.25984483663122,-2.82466872119205));
#65903=CARTESIAN_POINT('Ctrl Pts',(19.9961413776194,9.38641645673583,-2.80226300874746));
#65904=CARTESIAN_POINT('Ctrl Pts',(19.9889458669186,9.51297969810196,-2.77985877950743));
#65905=CARTESIAN_POINT('Ctrl Pts',(19.9817503562177,9.64055587871207,-2.76318290195909));
#65906=CARTESIAN_POINT('Ctrl Pts',(19.9745548455169,9.76861097645808,-2.75230319906341));
#65907=CARTESIAN_POINT('Ctrl Pts',(19.9673575905949,9.89669711528098,-2.74142085888347));
#65908=CARTESIAN_POINT('Ctrl Pts',(19.960160335673,10.0252620483062,-2.73633752911708));
#65909=CARTESIAN_POINT('Ctrl Pts',(19.9529630807511,10.1537676164009,-2.73706907365435));
#65910=CARTESIAN_POINT('Ctrl Pts',(19.9501644715859,10.2037362314554,-2.73735353033525));
#65911=CARTESIAN_POINT('Ctrl Pts',(19.9473658624208,10.2536958590512,-2.73851663601357));
#65912=CARTESIAN_POINT('Ctrl Pts',(19.9445672532556,10.3036148840483,-2.74055719522461));
#65913=CARTESIAN_POINT('Ctrl Pts',(19.9372997188826,10.4332465005499,-2.74585619673975));
#65914=CARTESIAN_POINT('Ctrl Pts',(19.9300321845096,10.5626553456609,-2.75707812798666));
#65915=CARTESIAN_POINT('Ctrl Pts',(19.9227646501365,10.6912947465663,-2.77417988282387));
#65916=CARTESIAN_POINT('Ctrl Pts',(19.91549833993,10.8199124790436,-2.79127875698733));
#65917=CARTESIAN_POINT('Ctrl Pts',(19.9082320297235,10.9477606866541,-2.81425543359745));
#65918=CARTESIAN_POINT('Ctrl Pts',(19.9009657195169,11.0742992481297,-2.84301510939317));
#65919=CARTESIAN_POINT('Ctrl Pts',(19.8936990472744,11.2008441142512,-2.87177621810837));
#65920=CARTESIAN_POINT('Ctrl Pts',(19.8864323750319,11.3260788692529,-2.90632082903432));
#65921=CARTESIAN_POINT('Ctrl Pts',(19.8791657027894,11.4494746488613,-2.94650324702691));
#65922=CARTESIAN_POINT('Ctrl Pts',(19.8718993416436,11.572865145719,-2.98668394475241));
#65923=CARTESIAN_POINT('Ctrl Pts',(19.8646329804978,11.6944164996854,-3.03250185894799));
#65924=CARTESIAN_POINT('Ctrl Pts',(19.857366619352,11.8136161997892,-3.08376180172764));
#65925=CARTESIAN_POINT('Ctrl Pts',(19.8500988473739,11.9328390436335,-3.13503169710623));
#65926=CARTESIAN_POINT('Ctrl Pts',(19.8428310753959,12.0497090072423,-3.19174559577496));
#65927=CARTESIAN_POINT('Ctrl Pts',(19.8355633034179,12.1637343634684,-3.25366051264916));
#65928=CARTESIAN_POINT('Ctrl Pts',(19.8331160717277,12.2021294130214,-3.27450873781707));
#65929=CARTESIAN_POINT('Ctrl Pts',(19.8306688400376,12.2402021300839,-3.29594627973528));
#65930=CARTESIAN_POINT('Ctrl Pts',(19.8282216083474,12.2779343732715,-3.31796269115241));
#65931=CARTESIAN_POINT('Ctrl Pts',(19.8209722370613,12.3897076236044,-3.3831813385709));
#65932=CARTESIAN_POINT('Ctrl Pts',(19.8137228657752,12.4985292694164,-3.45350511738675));
#65933=CARTESIAN_POINT('Ctrl Pts',(19.8064734944891,12.6039381989666,-3.52864225417559));
#65934=CARTESIAN_POINT('Ctrl Pts',(19.7992255471016,12.7093264244276,-3.60376463276527));
#65935=CARTESIAN_POINT('Ctrl Pts',(19.7919775997141,12.8113029891484,-3.68369828266069));
#65936=CARTESIAN_POINT('Ctrl Pts',(19.7847296523266,12.9094366941866,-3.76810876168227));
#65937=CARTESIAN_POINT('Ctrl Pts',(19.7774814460529,13.007573904419,-3.85252225572431));
#65938=CARTESIAN_POINT('Ctrl Pts',(19.7702332397791,13.1018677159777,-3.94141267555906));
#65939=CARTESIAN_POINT('Ctrl Pts',(19.7629850335054,13.1919206551921,-4.03440583851178));
#65940=CARTESIAN_POINT('Ctrl Pts',(19.7557371455646,13.2819696393849,-4.12739491731172));
#65941=CARTESIAN_POINT('Ctrl Pts',(19.7484892576238,13.3677778844239,-4.22448612893644));
#65942=CARTESIAN_POINT('Ctrl Pts',(19.7412413696829,13.4489855172323,-4.32526919094931));
#65943=CARTESIAN_POINT('Ctrl Pts',(19.7339919237521,13.5302106062536,-4.42607391706597));
#65944=CARTESIAN_POINT('Ctrl Pts',(19.7267424778214,13.6068328911244,-4.53057180878018));
#65945=CARTESIAN_POINT('Ctrl Pts',(19.7194930318906,13.6785332358806,-4.63832007024348));
#65946=CARTESIAN_POINT('Ctrl Pts',(19.7169540090735,13.7036453359045,-4.67605747762233));
#65947=CARTESIAN_POINT('Ctrl Pts',(19.7144149862564,13.7281540642729,-4.71419332453206));
#65948=CARTESIAN_POINT('Ctrl Pts',(19.7118759634392,13.7520469693732,-4.75270775049499));
#65949=CARTESIAN_POINT('Ctrl Pts',(19.7046273193903,13.820258709417,-4.86266240024108));
#65950=CARTESIAN_POINT('Ctrl Pts',(19.6973786753414,13.8834733182431,-4.97574546948885));
#65951=CARTESIAN_POINT('Ctrl Pts',(19.6901300312925,13.9414199126782,-5.09148340868428));
#65952=CARTESIAN_POINT('Ctrl Pts',(19.6828828572101,13.9993547560108,-5.20719787715811));
#65953=CARTESIAN_POINT('Ctrl Pts',(19.6756356831278,14.0520235610632,-5.3255658322583));
#65954=CARTESIAN_POINT('Ctrl Pts',(19.6683885090455,14.0992018473551,-5.44609001447772));
#65955=CARTESIAN_POINT('Ctrl Pts',(19.6611411361963,14.1463814275969,-5.56661750229129));
#65956=CARTESIAN_POINT('Ctrl Pts',(19.6538937633471,14.1880700584847,-5.68930101442326));
#65957=CARTESIAN_POINT('Ctrl Pts',(19.6466463904979,14.2240916631679,-5.81362395847015));
#65958=CARTESIAN_POINT('Ctrl Pts',(19.6393993687001,14.2601115230209,-5.93794088050801));
#65959=CARTESIAN_POINT('Ctrl Pts',(19.6321523469024,14.2904648110072,-6.06389674266133));
#65960=CARTESIAN_POINT('Ctrl Pts',(19.6249053251046,14.3150255733708,-6.19096064702689));
#65961=CARTESIAN_POINT('Ctrl Pts',(19.617656786201,14.3395914773327,-6.31805115120036));
#65962=CARTESIAN_POINT('Ctrl Pts',(19.6104082472974,14.3583623684871,-6.44624982084262));
#65963=CARTESIAN_POINT('Ctrl Pts',(19.6031597083938,14.3712635105564,-6.57501609381955));
#65964=CARTESIAN_POINT('Ctrl Pts',(19.6006165784395,14.3757898407971,-6.62019338682416));
#65965=CARTESIAN_POINT('Ctrl Pts',(19.5980734484853,14.379594106723,-6.66544048851997));
#65966=CARTESIAN_POINT('Ctrl Pts',(19.5955303185311,14.3826745937204,-6.71073390220859));
#65967=CARTESIAN_POINT('Ctrl Pts',(19.5882769321214,14.3914606026636,-6.83991748197387));
#65968=CARTESIAN_POINT('Ctrl Pts',(19.5810235457117,14.3943581882403,-6.96952423534298));
#65969=CARTESIAN_POINT('Ctrl Pts',(19.5737701593021,14.3913501125846,-7.09900817068766));
#65970=CARTESIAN_POINT('Ctrl Pts',(19.5665181595134,14.388342611979,-7.22846735274605));
#65971=CARTESIAN_POINT('Ctrl Pts',(19.5592661597248,14.3794317103126,-7.3578034186612));
#65972=CARTESIAN_POINT('Ctrl Pts',(19.5520141599362,14.364652272981,-7.4864711961294));
#65973=CARTESIAN_POINT('Ctrl Pts',(19.5447618877024,14.3498722804115,-7.6151438074243));
#65974=CARTESIAN_POINT('Ctrl Pts',(19.5375096154687,14.3292233474636,-7.74314773673032));
#65975=CARTESIAN_POINT('Ctrl Pts',(19.5302573432349,14.3027921585418,-7.86994342313364));
#65976=CARTESIAN_POINT('Ctrl Pts',(19.5230053926805,14.2763621419927,-7.99673348543143));
#65977=CARTESIAN_POINT('Ctrl Pts',(19.515753442126,14.2441504547407,-8.12231507444478));
#65978=CARTESIAN_POINT('Ctrl Pts',(19.5085014915715,14.2062947632617,-8.24615948347003));
#65979=CARTESIAN_POINT('Ctrl Pts',(19.5012480222094,14.1684311435003,-8.370029829769));
#65980=CARTESIAN_POINT('Ctrl Pts',(19.4939945528474,14.1249212600331,-8.49216193935917));
#65981=CARTESIAN_POINT('Ctrl Pts',(19.4867410834853,14.0759525550909,-8.6120425647037));
#65982=CARTESIAN_POINT('Ctrl Pts',(19.4842222801979,14.0589479289135,-8.65367170769003));
#65983=CARTESIAN_POINT('Ctrl Pts',(19.4817034769104,14.0412854766061,-8.69502951553451));
#65984=CARTESIAN_POINT('Ctrl Pts',(19.4791846736229,14.0229744084962,-8.73609505223213));
#65985=CARTESIAN_POINT('Ctrl Pts',(19.4719351256642,13.9702720132359,-8.8542887115877));
#65986=CARTESIAN_POINT('Ctrl Pts',(19.4646855777054,13.9121739978676,-8.97010247114962));
#65987=CARTESIAN_POINT('Ctrl Pts',(19.4574360297467,13.8489203073898,-9.08304622535753));
#65988=CARTESIAN_POINT('Ctrl Pts',(19.4501879283525,13.7856792384645,-9.19596744292739));
#65989=CARTESIAN_POINT('Ctrl Pts',(19.4429398269584,13.7172847155392,-9.30601949578961));
#65990=CARTESIAN_POINT('Ctrl Pts',(19.4356917255643,13.6440223508725,-9.41273737593164));
#65991=CARTESIAN_POINT('Ctrl Pts',(19.428443400293,13.5707577233001,-9.5194585523432));
#65992=CARTESIAN_POINT('Ctrl Pts',(19.4211950750217,13.492625146295,-9.62284506291008));
#65993=CARTESIAN_POINT('Ctrl Pts',(19.4139467497504,13.4099534015183,-9.72246110724593));
#65994=CARTESIAN_POINT('Ctrl Pts',(19.4066987635179,13.3272855236945,-9.82207249206305));
#65995=CARTESIAN_POINT('Ctrl Pts',(19.3994507772854,13.2400791250862,-9.91791349828917));
#65996=CARTESIAN_POINT('Ctrl Pts',(19.3922027910529,13.1487029610089,-10.0095817782933));
#65997=CARTESIAN_POINT('Ctrl Pts',(19.384953278128,13.0573075497507,-10.1012693670086));
#65998=CARTESIAN_POINT('Ctrl Pts',(19.3777037652031,12.961740863451,-10.1887822292906));
#65999=CARTESIAN_POINT('Ctrl Pts',(19.3704542522781,12.8624084057092,-10.2717549795185));
#66000=CARTESIAN_POINT('Ctrl Pts',(19.3679158444237,12.8276272702665,-10.3008077839022));
#66001=CARTESIAN_POINT('Ctrl Pts',(19.3653774365692,12.792384745242,-10.3293043021381));
#66002=CARTESIAN_POINT('Ctrl Pts',(19.3628390287147,12.7566992070898,-10.3572300079481));
#66003=CARTESIAN_POINT('Ctrl Pts',(19.355587325406,12.6547530463751,-10.4370079415306));
#66004=CARTESIAN_POINT('Ctrl Pts',(19.3483356220973,12.5491521538965,-10.5121531526707));
#66005=CARTESIAN_POINT('Ctrl Pts',(19.3410839187886,12.4403383965228,-10.582344889197));
#66006=CARTESIAN_POINT('Ctrl Pts',(19.3338336305964,12.3315458733526,-10.6525229283228));
#66007=CARTESIAN_POINT('Ctrl Pts',(19.3265833424042,12.2195420262118,-10.7177492338765));
#66008=CARTESIAN_POINT('Ctrl Pts',(19.319333054212,12.1047973069638,-10.7777466232003));
#66009=CARTESIAN_POINT('Ctrl Pts',(19.3120825180557,11.9900486633794,-10.8377460644699));
#66010=CARTESIAN_POINT('Ctrl Pts',(19.3048319818994,11.8725592649077,-10.8925160688187));
#66011=CARTESIAN_POINT('Ctrl Pts',(19.2975814457431,11.7528240201902,-10.9418254813568));
#66012=CARTESIAN_POINT('Ctrl Pts',(19.2903312406935,11.6330942433642,-10.9911326421057));
#66013=CARTESIAN_POINT('Ctrl Pts',(19.283081035644,11.5111191456424,-11.0349795799072));
#66014=CARTESIAN_POINT('Ctrl Pts',(19.2758308305944,11.3874132828957,-11.0731834199695));
#66015=CARTESIAN_POINT('Ctrl Pts',(19.2685791058577,11.2636814906467,-11.1113952677894));
#66016=CARTESIAN_POINT('Ctrl Pts',(19.2613273811211,11.1382185391783,-11.1439615539113));
#66017=CARTESIAN_POINT('Ctrl Pts',(19.2540756563844,11.0115541411716,-11.1707492722582));
#66018=CARTESIAN_POINT('Ctrl Pts',(19.2515482321917,10.9674081379115,-11.1800855239602));
#66019=CARTESIAN_POINT('Ctrl Pts',(19.2490208079991,10.9231163019457,-11.1887202965382));
#66020=CARTESIAN_POINT('Ctrl Pts',(19.2464933838065,10.8787013672108,-11.1966494148749));
#66021=CARTESIAN_POINT('Ctrl Pts',(19.2390336219372,10.7476094683813,-11.2200524252586));
#66022=CARTESIAN_POINT('Ctrl Pts',(19.231573860068,10.6154089528811,-11.2373107444924));
#66023=CARTESIAN_POINT('Ctrl Pts',(19.2241140981988,10.4826720229851,-11.2483453864041));
#66024=CARTESIAN_POINT('Ctrl Pts',(19.2175155086208,10.3652585535498,-11.2581061635431));
#66025=CARTESIAN_POINT('Ctrl Pts',(19.2109169190427,10.2474256436952,-11.2629979845103));
#66026=CARTESIAN_POINT('Ctrl Pts',(19.2043183294647,10.1295728822702,-11.262999999377));
#66027=CARTESIAN_POINT('Ctrl Pts',(19.2043183294109,10.1295728813087,-11.262999999377));
#66028=CARTESIAN_POINT('Ctrl Pts',(19.1970583189289,9.99990694692026,-11.2630022161781));
#66029=CARTESIAN_POINT('Ctrl Pts',(19.1897983084469,9.87023735638593,-11.2570840955062));
#66030=CARTESIAN_POINT('Ctrl Pts',(19.1825382979649,9.7411112248888,-11.2452706815193));
#66031=CARTESIAN_POINT('Ctrl Pts',(19.1752785223053,9.61198926992911,-11.233457649633));
#66032=CARTESIAN_POINT('Ctrl Pts',(19.1680187466457,9.48341108082839,-11.215749739548));
#66033=CARTESIAN_POINT('Ctrl Pts',(19.1607589709861,9.35591875974781,-11.1922238805591));
#66034=CARTESIAN_POINT('Ctrl Pts',(19.1534975256724,9.22839711708991,-11.1686926109282));
#66035=CARTESIAN_POINT('Ctrl Pts',(19.1462360803587,9.1019621791951,-11.1393407825559));
#66036=CARTESIAN_POINT('Ctrl Pts',(19.138974635045,8.97714636126784,-11.1042965403709));
#66037=CARTESIAN_POINT('Ctrl Pts',(19.1360323363295,8.92657166092885,-11.090096801295));
#66038=CARTESIAN_POINT('Ctrl Pts',(19.1330900376139,8.87626264874846,-11.0749630455192));
#66039=CARTESIAN_POINT('Ctrl Pts',(19.1301477388984,8.82625408154575,-11.0589061427966));
#66040=CARTESIAN_POINT('Ctrl Pts',(19.1264842468684,8.76398780436326,-11.0389134973053));
#66041=CARTESIAN_POINT('Ctrl Pts',(19.1228207548385,8.70217597612885,-11.0174859478408));
#66042=CARTESIAN_POINT('Ctrl Pts',(19.1191572628085,8.64088535679774,-10.9946458471364));
#66043=CARTESIAN_POINT('Origin',(23.734,10.1295,-7.));
#66044=CARTESIAN_POINT('',(17.734,8.64088535679774,-10.9946458471364));
#66045=CARTESIAN_POINT('',(18.0286142064722,8.64088528410776,-10.9946458200483));
#66046=CARTESIAN_POINT('',(23.734,8.64088535679774,-10.9946458471364));
#66047=CARTESIAN_POINT('',(17.7339050262067,5.86731958600617,-6.91641101407839));
#66048=CARTESIAN_POINT('Origin',(17.734,10.1295,-7.));
#66049=CARTESIAN_POINT('Ctrl Pts',(17.7339050262067,5.86731958600617,-6.91641101407839));
#66050=CARTESIAN_POINT('Ctrl Pts',(17.7472545315539,5.86268934162998,-7.15250595738485));
#66051=CARTESIAN_POINT('Ctrl Pts',(17.7606088204071,5.87768407296756,-7.38858354784552));
#66052=CARTESIAN_POINT('Ctrl Pts',(17.7867512045192,5.94579532231527,-7.8502465191533));
#66053=CARTESIAN_POINT('Ctrl Pts',(17.7995044918489,5.99788017560926,-8.07518560832005));
#66054=CARTESIAN_POINT('Ctrl Pts',(17.8350441223152,6.19253199136132,-8.68577563313481));
#66055=CARTESIAN_POINT('Ctrl Pts',(17.8582714071464,6.37296588560031,-9.05669361479852));
#66056=CARTESIAN_POINT('Ctrl Pts',(17.8967465912778,6.75751592584523,-9.62257240524602));
#66057=CARTESIAN_POINT('Ctrl Pts',(17.9119120419527,6.93290530427956,-9.8337166577424));
#66058=CARTESIAN_POINT('Ctrl Pts',(17.9585433380038,7.53005115412866,-10.4260456333765));
#66059=CARTESIAN_POINT('Ctrl Pts',(17.9907102178401,8.00846843554533,-10.7411421365182));
#66060=CARTESIAN_POINT('Ctrl Pts',(18.0243885125157,8.5697845022952,-10.9676068626257));
#66061=CARTESIAN_POINT('Ctrl Pts',(18.0265024679027,8.60524950852272,-10.9813660595043));
#66062=CARTESIAN_POINT('Ctrl Pts',(18.0286142064722,8.64088528410776,-10.9946458200483));
#66063=CARTESIAN_POINT('Origin',(-23.734,10.1295,-7.));
#66064=CARTESIAN_POINT('',(-18.0286142198359,11.618114722277,-10.994645817669));
#66065=CARTESIAN_POINT('',(-17.734,11.6181146495903,-10.9946458447559));
#66066=CARTESIAN_POINT('',(-23.734,11.6181146495903,-10.9946458447559));
#66067=CARTESIAN_POINT('',(-17.7339050342228,14.3916804139849,-6.91641101362462));
#66068=CARTESIAN_POINT('Origin',(-17.734,10.1295,-7.));
#66069=CARTESIAN_POINT('Ctrl Pts',(-17.7339050342228,14.3916804139849,-6.91641101362462));
#66070=CARTESIAN_POINT('Ctrl Pts',(-17.7472546703102,14.3963107039188,-7.15250827862387));
#66071=CARTESIAN_POINT('Ctrl Pts',(-17.7606090905621,14.3813156320825,-7.38858818646879));
#66072=CARTESIAN_POINT('Ctrl Pts',(-17.7867517208388,14.3132029843049,-7.85025542053381));
#66073=CARTESIAN_POINT('Ctrl Pts',(-17.799505122171,14.261117122435,-8.07519644101184));
#66074=CARTESIAN_POINT('Ctrl Pts',(-17.8350446877022,14.0664638141747,-8.68578459435684));
#66075=CARTESIAN_POINT('Ctrl Pts',(-17.8582717904186,13.8860307362702,-9.05669910101929));
#66076=CARTESIAN_POINT('Ctrl Pts',(-17.8967467678593,13.5014823080873,-9.62257466023843));
#66077=CARTESIAN_POINT('Ctrl Pts',(-17.9119122070986,13.3260928888101,-9.83371868146643));
#66078=CARTESIAN_POINT('Ctrl Pts',(-17.9585434935157,12.7289467612535,-10.4260472219077));
#66079=CARTESIAN_POINT('Ctrl Pts',(-17.990710378402,12.2505292507666,-10.7411434545049));
#66080=CARTESIAN_POINT('Ctrl Pts',(-18.024388625212,11.6892138344056,-10.9676075078961));
#66081=CARTESIAN_POINT('Ctrl Pts',(-18.0265025308825,11.6537496589754,-10.9813663696733));
#66082=CARTESIAN_POINT('Ctrl Pts',(-18.0286142198359,11.618114722277,-10.994645817669));
#66083=CARTESIAN_POINT('Origin',(-23.734,10.1295,-7.));
#66084=CARTESIAN_POINT('',(-19.5287463281039,11.618114650837,-10.9946458442913));
#66085=CARTESIAN_POINT('',(-19.1191572624809,11.6181146495903,-10.9946458447559));
#66086=CARTESIAN_POINT('',(-23.734,11.6181146495903,-10.9946458447559));
#66087=CARTESIAN_POINT('',(-17.734,9.60084442449481,-11.2300936493755));
#66088=CARTESIAN_POINT('Ctrl Pts',(-19.1191572624809,11.6181146495903,-10.9946458447559));
#66089=CARTESIAN_POINT('Ctrl Pts',(-19.1119070028363,11.7394122804076,-10.9494439827604));
#66090=CARTESIAN_POINT('Ctrl Pts',(-19.1046567431916,11.8586672520018,-10.898706644448));
#66091=CARTESIAN_POINT('Ctrl Pts',(-19.097406483547,11.9753756588468,-10.8426438882723));
#66092=CARTESIAN_POINT('Ctrl Pts',(-19.0901561762952,12.0920848320306,-10.7865807639736));
#66093=CARTESIAN_POINT('Ctrl Pts',(-19.0829058690433,12.2062470931261,-10.7251922967873));
#66094=CARTESIAN_POINT('Ctrl Pts',(-19.0756555617915,12.3173806376937,-10.658735753673));
#66095=CARTESIAN_POINT('Ctrl Pts',(-19.0684059351248,12.4285037501756,-10.5922854488224));
#66096=CARTESIAN_POINT('Ctrl Pts',(-19.061156308458,12.5365984180107,-10.5207681969686));
#66097=CARTESIAN_POINT('Ctrl Pts',(-19.0539066817912,12.6412096611553,-10.444485967174));
#66098=CARTESIAN_POINT('Ctrl Pts',(-19.0466552548783,12.7458468816354,-10.3681847947783));
#66099=CARTESIAN_POINT('Ctrl Pts',(-19.0394038279654,12.8469986686003,-10.2871164827276));
#66100=CARTESIAN_POINT('Ctrl Pts',(-19.0321524010525,12.9442407270079,-10.2016251560298));
#66101=CARTESIAN_POINT('Ctrl Pts',(-19.0260356320317,13.0262669568152,-10.1295109769896));
#66102=CARTESIAN_POINT('Ctrl Pts',(-19.0199188630109,13.1055117254018,-10.054250454771));
#66103=CARTESIAN_POINT('Ctrl Pts',(-19.0138020939901,13.1817396470563,-9.97607159472646));
#66104=CARTESIAN_POINT('Ctrl Pts',(-19.006551083536,13.2721026238059,-9.88339591422544));
#66105=CARTESIAN_POINT('Ctrl Pts',(-18.999300073082,13.3582578890542,-9.7865849347629));
#66106=CARTESIAN_POINT('Ctrl Pts',(-18.9920490626279,13.4398386609267,-9.68604299108816));
#66107=CARTESIAN_POINT('Ctrl Pts',(-18.9847994767659,13.5214034047821,-9.58552080069554));
#66108=CARTESIAN_POINT('Ctrl Pts',(-18.9775498909039,13.598395230372,-9.48126937662048));
#66109=CARTESIAN_POINT('Ctrl Pts',(-18.9703003050419,13.670487562286,-9.37372620235276));
#66110=CARTESIAN_POINT('Ctrl Pts',(-18.9630504780159,13.7425822924159,-9.26617945056504));
#66111=CARTESIAN_POINT('Ctrl Pts',(-18.9558006509899,13.8097770076549,-9.15534101487568));
#66112=CARTESIAN_POINT('Ctrl Pts',(-18.9485508239639,13.871788232083,-9.04167768955162));
#66113=CARTESIAN_POINT('Ctrl Pts',(-18.9413013300434,13.9337966073018,-8.92801958667901));
#66114=CARTESIAN_POINT('Ctrl Pts',(-18.9340518361228,13.9906218040944,-8.81153715811386));
#66115=CARTESIAN_POINT('Ctrl Pts',(-18.9268023422023,14.0420262078369,-8.69272197155634));
#66116=CARTESIAN_POINT('Ctrl Pts',(-18.9195513255415,14.0934414089613,-8.57388182813012));
#66117=CARTESIAN_POINT('Ctrl Pts',(-18.9123003088806,14.1394334060361,-8.45270826559124));
#66118=CARTESIAN_POINT('Ctrl Pts',(-18.9050492922198,14.179812512944,-8.32971333282391));
#66119=CARTESIAN_POINT('Ctrl Pts',(-18.9025183445072,14.1939067307684,-8.28678228490142));
#66120=CARTESIAN_POINT('Ctrl Pts',(-18.8999873967946,14.2073175453242,-8.24362948941841));
#66121=CARTESIAN_POINT('Ctrl Pts',(-18.8974564490819,14.2200383107599,-8.20027718807187));
#66122=CARTESIAN_POINT('Ctrl Pts',(-18.8902054209966,14.2564826145993,-8.07607519327786));
#66123=CARTESIAN_POINT('Ctrl Pts',(-18.8829543929113,14.2872725593705,-7.95018973113526));
#66124=CARTESIAN_POINT('Ctrl Pts',(-18.8757033648259,14.3122734063533,-7.8231498229993));
#66125=CARTESIAN_POINT('Ctrl Pts',(-18.8684537617915,14.3372693398978,-7.69613488212714));
#66126=CARTESIAN_POINT('Ctrl Pts',(-18.861204158757,14.3564783785018,-7.56796628686594));
#66127=CARTESIAN_POINT('Ctrl Pts',(-18.8539545557225,14.369816831984,-7.43918352017531));
#66128=CARTESIAN_POINT('Ctrl Pts',(-18.8467047123714,14.3831557276218,-7.31039648447218));
#66129=CARTESIAN_POINT('Ctrl Pts',(-18.8394548690202,14.3906236100164,-7.18099558012911));
#66130=CARTESIAN_POINT('Ctrl Pts',(-18.8322050256691,14.3921885964997,-7.05152600577627));
#66131=CARTESIAN_POINT('Ctrl Pts',(-18.8249555159603,14.3937535109613,-6.92206238969404));
#66132=CARTESIAN_POINT('Ctrl Pts',(-18.8177060062514,14.3894160704854,-6.79253045561143));
#66133=CARTESIAN_POINT('Ctrl Pts',(-18.8104564965426,14.379196515432,-6.66347581554241));
#66134=CARTESIAN_POINT('Ctrl Pts',(-18.8032054650126,14.3689748150839,-6.53439408425104));
#66135=CARTESIAN_POINT('Ctrl Pts',(-18.7959544334827,14.3528685617423,-6.40579019172858));
#66136=CARTESIAN_POINT('Ctrl Pts',(-18.7887034019527,14.3309499353665,-6.27820540275729));
#66137=CARTESIAN_POINT('Ctrl Pts',(-18.7861725360264,14.3232995611519,-6.23367380835046));
#66138=CARTESIAN_POINT('Ctrl Pts',(-18.7836416701,14.3149415512132,-6.1892663009137));
#66139=CARTESIAN_POINT('Ctrl Pts',(-18.7811108041737,14.3058804482948,-6.14500564264953));
#66140=CARTESIAN_POINT('Ctrl Pts',(-18.7738598726569,14.2799203861494,-6.01819884556579));
#66141=CARTESIAN_POINT('Ctrl Pts',(-18.76660894114,14.2481760638575,-5.89255238081223));
#66142=CARTESIAN_POINT('Ctrl Pts',(-18.7593580096232,14.2107761567794,-5.76859676299603));
#66143=CARTESIAN_POINT('Ctrl Pts',(-18.7521085029907,14.1733835991768,-5.64466550376387));
#66144=CARTESIAN_POINT('Ctrl Pts',(-18.7448589963582,14.1303377735899,-5.52242475946198));
#66145=CARTESIAN_POINT('Ctrl Pts',(-18.7376094897257,14.0818173597769,-5.40239038322671));
#66146=CARTESIAN_POINT('Ctrl Pts',(-18.7303597415627,14.0332953294174,-5.2823520078264));
#66147=CARTESIAN_POINT('Ctrl Pts',(-18.7231099933996,13.9792984725236,-5.16452046926666));
#66148=CARTESIAN_POINT('Ctrl Pts',(-18.7158602452366,13.9200539214188,-5.04939241034578));
#66149=CARTESIAN_POINT('Ctrl Pts',(-18.7086108297512,13.860812088938,-4.93426963444092));
#66150=CARTESIAN_POINT('Ctrl Pts',(-18.7013614142658,13.7963232036895,-4.82185039661095));
#66151=CARTESIAN_POINT('Ctrl Pts',(-18.6941119987804,13.7268606462205,-4.71260729628162));
#66152=CARTESIAN_POINT('Ctrl Pts',(-18.6868610592732,13.6573834858556,-4.60334123011747));
#66153=CARTESIAN_POINT('Ctrl Pts',(-18.6796101197659,13.5829307508601,-4.4972529265802));
#66154=CARTESIAN_POINT('Ctrl Pts',(-18.6723591802586,13.5038196785847,-4.39478682125318));
#66155=CARTESIAN_POINT('Ctrl Pts',(-18.6698278399276,13.4762015957584,-4.35901537608866));
#66156=CARTESIAN_POINT('Ctrl Pts',(-18.6672964995966,13.448016156806,-4.32368511023057));
#66157=CARTESIAN_POINT('Ctrl Pts',(-18.6647651592655,13.4192780434162,-4.28881401872603));
#66158=CARTESIAN_POINT('Ctrl Pts',(-18.6575139795992,13.3369559546373,-4.18892363790238));
#66159=CARTESIAN_POINT('Ctrl Pts',(-18.650262799933,13.2500660974698,-4.09276745063653));
#66160=CARTESIAN_POINT('Ctrl Pts',(-18.6430116202667,13.1589706262765,-4.00075397399144));
#66161=CARTESIAN_POINT('Ctrl Pts',(-18.6357618651641,13.0678930516613,-3.9087585742755));
#66162=CARTESIAN_POINT('Ctrl Pts',(-18.6285121100615,12.9726117542656,-3.82090450717327));
#66163=CARTESIAN_POINT('Ctrl Pts',(-18.621262354959,12.8735262051464,-3.73756391856177));
#66164=CARTESIAN_POINT('Ctrl Pts',(-18.6140123603528,12.7744373826274,-3.65422057670254));
#66165=CARTESIAN_POINT('Ctrl Pts',(-18.6067623657466,12.671544319424,-3.57539123658429));
#66166=CARTESIAN_POINT('Ctrl Pts',(-18.5995123711404,12.565280302068,-3.50140838049687));
#66167=CARTESIAN_POINT('Ctrl Pts',(-18.5922627110611,12.4590211879107,-3.42742893810165));
#66168=CARTESIAN_POINT('Ctrl Pts',(-18.5850130509817,12.3493917154141,-3.35829572848366));
#66169=CARTESIAN_POINT('Ctrl Pts',(-18.5777633909024,12.2368547762457,-3.29429833269943));
#66170=CARTESIAN_POINT('Ctrl Pts',(-18.5705122115537,12.1242942533625,-3.23028752535143));
#66171=CARTESIAN_POINT('Ctrl Pts',(-18.5632610322051,12.0088253476332,-3.17141485196072));
#66172=CARTESIAN_POINT('Ctrl Pts',(-18.5560098528564,11.8909365133965,-3.11792447146199));
#66173=CARTESIAN_POINT('Ctrl Pts',(-18.5534797400234,11.8498022319187,-3.0992603767491));
#66174=CARTESIAN_POINT('Ctrl Pts',(-18.5509496271904,11.8083735322816,-3.08125114867534));
#66175=CARTESIAN_POINT('Ctrl Pts',(-18.5484195143573,11.7666717816433,-3.06390579922293));
#66176=CARTESIAN_POINT('Ctrl Pts',(-18.5411687398128,11.6471632806606,-3.01419765315347));
#66177=CARTESIAN_POINT('Ctrl Pts',(-18.5339179652682,11.5253676687474,-2.96992735828438));
#66178=CARTESIAN_POINT('Ctrl Pts',(-18.5266671907236,11.4017961818643,-2.93128626890347));
#66179=CARTESIAN_POINT('Ctrl Pts',(-18.5194178411145,11.2782489794753,-2.89265277333995));
#66180=CARTESIAN_POINT('Ctrl Pts',(-18.5121684915053,11.1529269281156,-2.85964637962311));
#66181=CARTESIAN_POINT('Ctrl Pts',(-18.5049191418962,11.0263572046861,-2.83240883070295));
#66182=CARTESIAN_POINT('Ctrl Pts',(-18.4976695492601,10.8997832381373,-2.80517036867211));
#66183=CARTESIAN_POINT('Ctrl Pts',(-18.490419956624,10.7719618531677,-2.78370121420388));
#66184=CARTESIAN_POINT('Ctrl Pts',(-18.4831703639879,10.6434315319627,-2.76809222921216));
#66185=CARTESIAN_POINT('Ctrl Pts',(-18.4759211027388,10.5149070860224,-2.75248395772461));
#66186=CARTESIAN_POINT('Ctrl Pts',(-18.4686718414897,10.3856741121022,-2.74273535980208));
#66187=CARTESIAN_POINT('Ctrl Pts',(-18.4614225802406,10.2562771601344,-2.73888552704011));
#66188=CARTESIAN_POINT('Ctrl Pts',(-18.4541717917954,10.1268529482137,-2.73503488323693));
#66189=CARTESIAN_POINT('Ctrl Pts',(-18.4469210033502,9.99726503491748,-2.73708549638287));
#66190=CARTESIAN_POINT('Ctrl Pts',(-18.439670214905,9.86805928547783,-2.74502435344336));
#66191=CARTESIAN_POINT('Ctrl Pts',(-18.4371380997531,9.82293814612162,-2.74779675542476));
#66192=CARTESIAN_POINT('Ctrl Pts',(-18.4346059846011,9.77786359757213,-2.75128678775841));
#66193=CARTESIAN_POINT('Ctrl Pts',(-18.4320738694491,9.73285879557307,-2.75549240135552));
#66194=CARTESIAN_POINT('Ctrl Pts',(-18.4248227518998,9.60398033231389,-2.76753584990727));
#66195=CARTESIAN_POINT('Ctrl Pts',(-18.4175716343504,9.47562755644352,-2.78545561278176));
#66196=CARTESIAN_POINT('Ctrl Pts',(-18.410320516801,9.34834184038334,-2.80918135328379));
#66197=CARTESIAN_POINT('Ctrl Pts',(-18.4030708252718,9.22108115660127,-2.83290242783151));
#66198=CARTESIAN_POINT('Ctrl Pts',(-18.3958211337425,9.09488745366868,-2.86242713899534));
#66199=CARTESIAN_POINT('Ctrl Pts',(-18.3885714422132,8.97029295673026,-2.89763384973576));
#66200=CARTESIAN_POINT('Ctrl Pts',(-18.3813215126581,8.84569436903645,-2.93284171640238));
#66201=CARTESIAN_POINT('Ctrl Pts',(-18.3740715831029,8.72269542589954,-2.97373186495665));
#66202=CARTESIAN_POINT('Ctrl Pts',(-18.3668216535478,8.60181451476024,-3.02013240695274));
#66203=CARTESIAN_POINT('Ctrl Pts',(-18.3595720591937,8.48093919255952,-3.06653080361607));
#66204=CARTESIAN_POINT('Ctrl Pts',(-18.3523224648397,8.36218202856164,-3.11843895858724));
#66205=CARTESIAN_POINT('Ctrl Pts',(-18.3450728704856,8.24604252945651,-3.17563639847701));
#66206=CARTESIAN_POINT('Ctrl Pts',(-18.3378217572843,8.1298786982106,-3.23284582168142));
#66207=CARTESIAN_POINT('Ctrl Pts',(-18.3305706440831,8.01633393716156,-3.29534658989738));
#66208=CARTESIAN_POINT('Ctrl Pts',(-18.3233195308819,7.90588451646996,-3.36287157479895));
#66209=CARTESIAN_POINT('Ctrl Pts',(-18.3207890954349,7.8673407616755,-3.38643590355911));
#66210=CARTESIAN_POINT('Ctrl Pts',(-18.3182586599879,7.82917373057229,-3.41061168551164));
#66211=CARTESIAN_POINT('Ctrl Pts',(-18.3157282245409,7.79140288446141,-3.43538629325559));
#66212=CARTESIAN_POINT('Ctrl Pts',(-18.3084765678271,7.68316016674423,-3.50638472587502));
#66213=CARTESIAN_POINT('Ctrl Pts',(-18.3012249111132,7.57813431895171,-3.58232985338498));
#66214=CARTESIAN_POINT('Ctrl Pts',(-18.2939732543993,7.47677079571313,-3.66290593948514));
#66215=CARTESIAN_POINT('Ctrl Pts',(-18.2867230174911,7.37542711849153,-3.74346624955146));
#66216=CARTESIAN_POINT('Ctrl Pts',(-18.2794727805829,7.27774460581844,-3.82865549458475));
#66217=CARTESIAN_POINT('Ctrl Pts',(-18.2722225436747,7.18413660431221,-3.91811689589912));
#66218=CARTESIAN_POINT('Ctrl Pts',(-18.2649720651783,7.09052548365482,-4.00758127819406));
#66219=CARTESIAN_POINT('Ctrl Pts',(-18.2577215866819,7.00098939780611,-4.10131786511218));
#66220=CARTESIAN_POINT('Ctrl Pts',(-18.2504711081855,6.91590593318733,-4.19893195838688));
#66221=CARTESIAN_POINT('Ctrl Pts',(-18.2432209643435,6.8308263956953,-4.296541546169));
#66222=CARTESIAN_POINT('Ctrl Pts',(-18.2359708205014,6.75019929407812,-4.39802802065957));
#66223=CARTESIAN_POINT('Ctrl Pts',(-18.2287206766593,6.67436277978478,-4.5029625975001));
#66224=CARTESIAN_POINT('Ctrl Pts',(-18.2214690178202,6.5985104186205,-4.6079191015707));
#66225=CARTESIAN_POINT('Ctrl Pts',(-18.2142173589811,6.52745084621281,-4.71632486665446));
#66226=CARTESIAN_POINT('Ctrl Pts',(-18.206965700142,6.46147983464391,-4.82772076690378));
#66227=CARTESIAN_POINT('Ctrl Pts',(-18.2044379933056,6.43848435448568,-4.86654997617272));
#66228=CARTESIAN_POINT('Ctrl Pts',(-18.2019102864692,6.41610674542311,-4.90574224142944));
#66229=CARTESIAN_POINT('Ctrl Pts',(-18.1993825796327,6.39435825302684,-4.94527735934548));
#66230=CARTESIAN_POINT('Ctrl Pts',(-18.1921344615983,6.33199515075258,-5.05864303808309));
#66231=CARTESIAN_POINT('Ctrl Pts',(-18.1848863435638,6.27478555423617,-5.17487082656046));
#66232=CARTESIAN_POINT('Ctrl Pts',(-18.1776382255294,6.22297508950893,-5.29347366744233));
#66233=CARTESIAN_POINT('Ctrl Pts',(-18.1703915452606,6.17117490211235,-5.41205298179112));
#66234=CARTESIAN_POINT('Ctrl Pts',(-18.1631448649917,6.12477184866148,-5.53300609161682));
#66235=CARTESIAN_POINT('Ctrl Pts',(-18.1558981847229,6.08396397100318,-5.65582469964344));
#66236=CARTESIAN_POINT('Ctrl Pts',(-18.1486512534106,6.04315467965562,-5.77864756242078));
#66237=CARTESIAN_POINT('Ctrl Pts',(-18.1414043220982,6.00794106410452,-5.90333572510643));
#66238=CARTESIAN_POINT('Ctrl Pts',(-18.1341573907859,5.97847181466648,-6.02936412359387));
#66239=CARTESIAN_POINT('Ctrl Pts',(-18.126910778967,5.94900386443136,-6.15538696590101));
#66240=CARTESIAN_POINT('Ctrl Pts',(-18.1196641671482,5.92527985076615,-6.28274958823024));
#66241=CARTESIAN_POINT('Ctrl Pts',(-18.1124175553294,5.90739765777448,-6.4109152762346));
#66242=CARTESIAN_POINT('Ctrl Pts',(-18.1051693767042,5.88951159843356,-6.53910867523119));
#66243=CARTESIAN_POINT('Ctrl Pts',(-18.0979211980791,5.87746992980869,-6.66810514361617));
#66244=CARTESIAN_POINT('Ctrl Pts',(-18.090673019454,5.87131888145374,-6.79736100657538));
#66245=CARTESIAN_POINT('Ctrl Pts',(-18.0881276578775,5.86915880194306,-6.8427521212444));
#66246=CARTESIAN_POINT('Ctrl Pts',(-18.085582296301,5.8677246979414,-6.88817518983173));
#66247=CARTESIAN_POINT('Ctrl Pts',(-18.0830369347245,5.86701704802671,-6.93360659568108));
#66248=CARTESIAN_POINT('Ctrl Pts',(-18.075778159349,5.86499899612295,-7.06316633017908));
#66249=CARTESIAN_POINT('Ctrl Pts',(-18.0685193839736,5.86889196438214,-7.19284036543872));
#66250=CARTESIAN_POINT('Ctrl Pts',(-18.0612606085981,5.87868451109096,-7.32208178969175));
#66251=CARTESIAN_POINT('Ctrl Pts',(-18.0540032283321,5.8884751757089,-7.45129837422593));
#66252=CARTESIAN_POINT('Ctrl Pts',(-18.0467458480661,5.90416313081031,-7.58008217059496));
#66253=CARTESIAN_POINT('Ctrl Pts',(-18.0394884678001,5.92568494599538,-7.70788981609017));
#66254=CARTESIAN_POINT('Ctrl Pts',(-18.0322308822655,5.94720736990625,-7.83570107651326));
#66255=CARTESIAN_POINT('Ctrl Pts',(-18.0249732967308,5.97456393001379,-7.96253579089963));
#66256=CARTESIAN_POINT('Ctrl Pts',(-18.0177157111962,6.00763974228285,-8.08785891357838));
#66257=CARTESIAN_POINT('Ctrl Pts',(-18.0104585011979,6.04071384307759,-8.21317555153937));
#66258=CARTESIAN_POINT('Ctrl Pts',(-18.0032012911997,6.07950651480405,-8.33698042184617));
#66259=CARTESIAN_POINT('Ctrl Pts',(-17.9959440812014,6.12385252539537,-8.45875196973082));
#66260=CARTESIAN_POINT('Ctrl Pts',(-17.9886854754884,6.16820706466122,-8.58054693685623));
#66261=CARTESIAN_POINT('Ctrl Pts',(-17.9814268697753,6.21811695780158,-8.70030747718995));
#66262=CARTESIAN_POINT('Ctrl Pts',(-17.9741682640623,6.27336806870438,-8.81753006259657));
#66263=CARTESIAN_POINT('Ctrl Pts',(-17.9716759393136,6.29233916543256,-8.85777976925658));
#66264=CARTESIAN_POINT('Ctrl Pts',(-17.969183614565,6.31193956155937,-8.89773043939557));
#66265=CARTESIAN_POINT('Ctrl Pts',(-17.9666912898163,6.33215930540418,-8.93736229166527));
#66266=CARTESIAN_POINT('Ctrl Pts',(-17.9594570419305,6.39084934539216,-9.05239812062335));
#66267=CARTESIAN_POINT('Ctrl Pts',(-17.9522227940446,6.45478200713309,-9.1647874961122));
#66268=CARTESIAN_POINT('Ctrl Pts',(-17.9449885461588,6.52369336922076,-9.27405530746912));
#66269=CARTESIAN_POINT('Ctrl Pts',(-17.9377557403836,6.59259099417794,-9.38330133684209));
#66270=CARTESIAN_POINT('Ctrl Pts',(-17.9305229346084,6.66646515380628,-9.48942674829286));
#66271=CARTESIAN_POINT('Ctrl Pts',(-17.9232901288331,6.74500762221501,-9.59198386274208));
#66272=CARTESIAN_POINT('Ctrl Pts',(-17.9160569412351,6.82355423691301,-9.69454639122362));
#66273=CARTESIAN_POINT('Ctrl Pts',(-17.9088237536371,6.90676944361806,-9.79353996699944));
#66274=CARTESIAN_POINT('Ctrl Pts',(-17.9015905660391,6.99430342483591,-9.88854832659579));
#66275=CARTESIAN_POINT('Ctrl Pts',(-17.8943575860858,7.08183489319576,-9.98355395876547));
#66276=CARTESIAN_POINT('Ctrl Pts',(-17.8871246061326,7.17368464971698,-10.0745743487264));
#66277=CARTESIAN_POINT('Ctrl Pts',(-17.8798916261793,7.26946473159495,-10.1612287584861));
#66278=CARTESIAN_POINT('Ctrl Pts',(-17.8726568022711,7.36526923137027,-10.2479052596705));
#66279=CARTESIAN_POINT('Ctrl Pts',(-17.8654219783628,7.46500579836938,-10.3302133240362));
#66280=CARTESIAN_POINT('Ctrl Pts',(-17.8581871544545,7.56825173400053,-10.4078110745631));
#66281=CARTESIAN_POINT('Ctrl Pts',(-17.8555733179391,7.60555298694718,-10.4358460117526));
#66282=CARTESIAN_POINT('Ctrl Pts',(-17.8529594814236,7.64331200171484,-10.4632665119052));
#66283=CARTESIAN_POINT('Ctrl Pts',(-17.8503456449081,7.68150784529143,-10.4900577947199));
#66284=CARTESIAN_POINT('Ctrl Pts',(-17.8430549103876,7.7880469320545,-10.5647863132449));
#66285=CARTESIAN_POINT('Ctrl Pts',(-17.835764175867,7.89802714309815,-10.6346446939616));
#66286=CARTESIAN_POINT('Ctrl Pts',(-17.8284734413464,8.01098544471159,-10.6993330586784));
#66287=CARTESIAN_POINT('Ctrl Pts',(-17.8211842251912,8.12392022167701,-10.7640079514238));
#66288=CARTESIAN_POINT('Ctrl Pts',(-17.8138950090359,8.23983155880657,-10.8235148084672));
#66289=CARTESIAN_POINT('Ctrl Pts',(-17.8066057928806,8.35823017917576,-10.8775987700944));
#66290=CARTESIAN_POINT('Ctrl Pts',(-17.7993168960918,8.47662361207955,-10.9316803621104));
#66291=CARTESIAN_POINT('Ctrl Pts',(-17.7920279993031,8.59750380479902,-10.9803393896484));
#66292=CARTESIAN_POINT('Ctrl Pts',(-17.7847391025143,8.72035948000763,-11.0233682400342));
#66293=CARTESIAN_POINT('Ctrl Pts',(-17.777450984006,8.84320203715903,-11.0663924959646));
#66294=CARTESIAN_POINT('Ctrl Pts',(-17.7701628654976,8.96801933638021,-11.1037876646716));
#66295=CARTESIAN_POINT('Ctrl Pts',(-17.7628747469893,9.09428288699931,-11.1353953292219));
#66296=CARTESIAN_POINT('Ctrl Pts',(-17.7555860914211,9.22055574195172,-11.1670053229341));
#66297=CARTESIAN_POINT('Ctrl Pts',(-17.7482974358529,9.34827473355606,-11.1928268781538));
#66298=CARTESIAN_POINT('Ctrl Pts',(-17.7410087802847,9.47689872479612,-11.2127521379263));
#66299=CARTESIAN_POINT('Ctrl Pts',(-17.7386725201898,9.51812705492797,-11.2191388561422));
#66300=CARTESIAN_POINT('Ctrl Pts',(-17.7363362600949,9.55944829064432,-11.2249201712499));
#66301=CARTESIAN_POINT('Ctrl Pts',(-17.734,9.6008444244948,-11.2300936493755));
#66302=CARTESIAN_POINT('Origin',(-17.734,10.1295,-7.));
#66303=CARTESIAN_POINT('Ctrl Pts',(-18.0286142198359,11.618114722277,-10.994645817669));
#66304=CARTESIAN_POINT('Ctrl Pts',(-18.0397899417923,11.4295234319622,-11.0649248321473));
#66305=CARTESIAN_POINT('Ctrl Pts',(-18.0508912348905,11.2361487040778,-11.1217763475609));
#66306=CARTESIAN_POINT('Ctrl Pts',(-18.0855390992679,10.6302068195219,-11.2541656503512));
#66307=CARTESIAN_POINT('Ctrl Pts',(-18.1093855857369,10.2100253826391,-11.2827745919004));
#66308=CARTESIAN_POINT('Ctrl Pts',(-18.1471820760258,9.53442686787758,-11.2291898906281));
#66309=CARTESIAN_POINT('Ctrl Pts',(-18.1614172796559,9.27881522463706,-11.1852708984346));
#66310=CARTESIAN_POINT('Ctrl Pts',(-18.190622001046,8.77281474633276,-11.0500330431345));
#66311=CARTESIAN_POINT('Ctrl Pts',(-18.2056655138667,8.52380028392084,-10.9579139355769));
#66312=CARTESIAN_POINT('Ctrl Pts',(-18.2520857621324,7.78229449195763,-10.6020365091));
#66313=CARTESIAN_POINT('Ctrl Pts',(-18.2822658968775,7.33181572759219,-10.2645063028337));
#66314=CARTESIAN_POINT('Ctrl Pts',(-18.3295643900168,6.77226297682638,-9.6420119018166));
#66315=CARTESIAN_POINT('Ctrl Pts',(-18.3453631324316,6.60632476873529,-9.41630116393842));
#66316=CARTESIAN_POINT('Ctrl Pts',(-18.3745510922519,6.33970460921812,-8.96713091919617));
#66317=CARTESIAN_POINT('Ctrl Pts',(-18.3879438485495,6.23381129189303,-8.74807419247257));
#66318=CARTESIAN_POINT('Ctrl Pts',(-18.4231083478773,6.00795504093371,-8.15680262527249));
#66319=CARTESIAN_POINT('Ctrl Pts',(-18.4452893358322,5.91943710373188,-7.77503571946316));
#66320=CARTESIAN_POINT('Ctrl Pts',(-18.4823846590503,5.85951254984844,-7.1169598782444));
#66321=CARTESIAN_POINT('Ctrl Pts',(-18.4973479370614,5.86070190714408,-6.84560128227382));
#66322=CARTESIAN_POINT('Ctrl Pts',(-18.5347901270604,5.92780682615062,-6.17395386811052));
#66323=CARTESIAN_POINT('Ctrl Pts',(-18.5577037975171,6.02500291571947,-5.77948263353823));
#66324=CARTESIAN_POINT('Ctrl Pts',(-18.611839791862,6.38541099251693,-4.88640861831262));
#66325=CARTESIAN_POINT('Ctrl Pts',(-18.6422260281472,6.69442287471882,-4.41432819085399));
#66326=CARTESIAN_POINT('Ctrl Pts',(-18.7055320907897,7.4779313868878,-3.61529311894462));
#66327=CARTESIAN_POINT('Ctrl Pts',(-18.735995631186,7.94522306179521,-3.29648992480263));
#66328=CARTESIAN_POINT('Ctrl Pts',(-18.7812358479547,8.68608970371472,-2.98133201949152));
#66329=CARTESIAN_POINT('Ctrl Pts',(-18.7951410857659,8.91925017279069,-2.9050736050566));
#66330=CARTESIAN_POINT('Ctrl Pts',(-18.8352496726883,9.6127897355547,-2.74269183357329));
#66331=CARTESIAN_POINT('Ctrl Pts',(-18.8606371003608,10.0823473599482,-2.71170941554586));
#66332=CARTESIAN_POINT('Ctrl Pts',(-18.9017618534194,10.8091993674334,-2.78332875356657));
#66333=CARTESIAN_POINT('Ctrl Pts',(-18.9166851645012,11.0679300498758,-2.8332674363393));
#66334=CARTESIAN_POINT('Ctrl Pts',(-18.9543381615285,11.7116484510719,-3.02055286889724));
#66335=CARTESIAN_POINT('Ctrl Pts',(-18.9765376750217,12.0845440079559,-3.18988324934561));
#66336=CARTESIAN_POINT('Ctrl Pts',(-19.0125999013546,12.6253538391597,-3.53605033808907));
#66337=CARTESIAN_POINT('Ctrl Pts',(-19.0259253745705,12.8122090384483,-3.67865896236762));
#66338=CARTESIAN_POINT('Ctrl Pts',(-19.0711062246202,13.4071505539574,-4.21583690391118));
#66339=CARTESIAN_POINT('Ctrl Pts',(-19.1018264230492,13.7479366700916,-4.67589507881516));
#66340=CARTESIAN_POINT('Ctrl Pts',(-19.1493255902435,14.1047108978616,-5.43622809776405));
#66341=CARTESIAN_POINT('Ctrl Pts',(-19.1647081333843,14.1966683223724,-5.69392415695462));
#66342=CARTESIAN_POINT('Ctrl Pts',(-19.2024932025121,14.3622053978055,-6.35105363367153));
#66343=CARTESIAN_POINT('Ctrl Pts',(-19.2246636397218,14.4046789399255,-6.75553616149174));
#66344=CARTESIAN_POINT('Ctrl Pts',(-19.2628448806025,14.3793616086868,-7.42998982348097));
#66345=CARTESIAN_POINT('Ctrl Pts',(-19.278113450657,14.3435617867383,-7.69850243303745));
#66346=CARTESIAN_POINT('Ctrl Pts',(-19.3145998245686,14.196207970448,-8.33476912891735));
#66347=CARTESIAN_POINT('Ctrl Pts',(-19.335512893636,14.0599945188133,-8.69438243891843));
#66348=CARTESIAN_POINT('Ctrl Pts',(-19.3695475245382,13.772450891264,-9.22503986555262));
#66349=CARTESIAN_POINT('Ctrl Pts',(-19.3820444339168,13.6523714961616,-9.41065803948714));
#66350=CARTESIAN_POINT('Ctrl Pts',(-19.4101330724861,13.3490093207116,-9.80819322705906));
#66351=CARTESIAN_POINT('Ctrl Pts',(-19.4255790255469,13.1581441494962,-10.0130563185497));
#66352=CARTESIAN_POINT('Ctrl Pts',(-19.4697727609324,12.5604719313637,-10.5399554439652));
#66353=CARTESIAN_POINT('Ctrl Pts',(-19.4992177593519,12.1132641842266,-10.8086187469988));
#66354=CARTESIAN_POINT('Ctrl Pts',(-19.5283177970268,11.6253074398653,-10.991959899824));
#66355=CARTESIAN_POINT('Ctrl Pts',(-19.5285320816716,11.6217118974251,-10.9933053214558));
#66356=CARTESIAN_POINT('Ctrl Pts',(-19.5287463281039,11.618114650837,-10.9946458442913));
#66357=CARTESIAN_POINT('Origin',(-23.734,10.1295,-7.));
#66358=CARTESIAN_POINT('',(-21.0285562874006,11.6181146495903,-10.9946458447559));
#66359=CARTESIAN_POINT('',(-20.6190482780298,11.6181146495903,-10.9946458447559));
#66360=CARTESIAN_POINT('',(-23.734,11.6181146495903,-10.9946458447559));
#66361=CARTESIAN_POINT('',(-19.2043183294647,10.1294271144268,-11.2629999993769));
#66362=CARTESIAN_POINT('Ctrl Pts',(-20.6190482780298,11.6181146495903,-10.9946458447559));
#66363=CARTESIAN_POINT('Ctrl Pts',(-20.6121906290549,11.7332039726838,-10.9517575239819));
#66364=CARTESIAN_POINT('Ctrl Pts',(-20.60533298008,11.8464456215055,-10.9038886682126));
#66365=CARTESIAN_POINT('Ctrl Pts',(-20.5984753311051,11.9573848895994,-10.8512343255603));
#66366=CARTESIAN_POINT('Ctrl Pts',(-20.5916138715458,12.06838580323,-10.7985507245105));
#66367=CARTESIAN_POINT('Ctrl Pts',(-20.5847524119864,12.1770814109274,-10.7410764995601));
#66368=CARTESIAN_POINT('Ctrl Pts',(-20.5778909524271,12.2830397599629,-10.6790536150291));
#66369=CARTESIAN_POINT('Ctrl Pts',(-20.5710273823149,12.3890307012904,-10.6170116525494));
#66370=CARTESIAN_POINT('Ctrl Pts',(-20.5641638122027,12.4922823613388,-10.5504184614062));
#66371=CARTESIAN_POINT('Ctrl Pts',(-20.5573002420905,12.5923911973628,-10.4795597350747));
#66372=CARTESIAN_POINT('Ctrl Pts',(-20.5504294658789,12.6926051381959,-10.4086266137826));
#66373=CARTESIAN_POINT('Ctrl Pts',(-20.5435586896673,12.7896693412134,-10.3334192620168));
#66374=CARTESIAN_POINT('Ctrl Pts',(-20.5366879134557,12.8832127424892,-10.2542641459864));
#66375=CARTESIAN_POINT('Ctrl Pts',(-20.533223768236,12.9303759619541,-10.2143552902232));
#66376=CARTESIAN_POINT('Ctrl Pts',(-20.5297596230163,12.9766447457956,-10.1734435061821));
#66377=CARTESIAN_POINT('Ctrl Pts',(-20.5262954777966,13.0219751493983,-10.1315741265557));
#66378=CARTESIAN_POINT('Ctrl Pts',(-20.5192445844224,13.1142402890342,-10.0463535273403));
#66379=CARTESIAN_POINT('Ctrl Pts',(-20.5121936910481,13.202815074995,-9.95697931960131));
#66380=CARTESIAN_POINT('Ctrl Pts',(-20.5051427976739,13.2873186628024,-9.86379997430979));
#66381=CARTESIAN_POINT('Ctrl Pts',(-20.4980972350301,13.3717583628408,-9.77069107597379));
#66382=CARTESIAN_POINT('Ctrl Pts',(-20.4910516723863,13.4521327375992,-9.67378305102304));
#66383=CARTESIAN_POINT('Ctrl Pts',(-20.4840061097425,13.5280976244367,-9.57346132420387));
#66384=CARTESIAN_POINT('Ctrl Pts',(-20.4769645310387,13.6040195566425,-9.47319632468334));
#66385=CARTESIAN_POINT('Ctrl Pts',(-20.4699229523349,13.6755367369793,-9.36952177262488));
#66386=CARTESIAN_POINT('Ctrl Pts',(-20.462881373631,13.7423453554112,-9.26285603560717));
#66387=CARTESIAN_POINT('Ctrl Pts',(-20.4558422186787,13.8091309779363,-9.15622701354339));
#66388=CARTESIAN_POINT('Ctrl Pts',(-20.4488030637263,13.8712110646756,-9.04660918159906));
#66389=CARTESIAN_POINT('Ctrl Pts',(-20.4417639087739,13.9283253559476,-8.93444951213759));
#66390=CARTESIAN_POINT('Ctrl Pts',(-20.4347249074765,13.9854384004943,-8.82229229096549));
#66391=CARTESIAN_POINT('Ctrl Pts',(-20.4276859061791,14.0375856880425,-8.7075936815819));
#66392=CARTESIAN_POINT('Ctrl Pts',(-20.4206469048817,14.0845531721528,-8.59082475635887));
#66393=CARTESIAN_POINT('Ctrl Pts',(-20.4170812142173,14.1083451154338,-8.53167405458023));
#66394=CARTESIAN_POINT('Ctrl Pts',(-20.4135155235529,14.1308086464159,-8.47199245138789));
#66395=CARTESIAN_POINT('Ctrl Pts',(-20.4099498328884,14.1519206685263,-8.41184310934763));
#66396=CARTESIAN_POINT('Ctrl Pts',(-20.4023577742973,14.1968723269634,-8.28377329848487));
#66397=CARTESIAN_POINT('Ctrl Pts',(-20.3947657157062,14.235676866179,-8.15363107788822));
#66398=CARTESIAN_POINT('Ctrl Pts',(-20.387173657115,14.2681822825818,-8.02199704688589));
#66399=CARTESIAN_POINT('Ctrl Pts',(-20.3793762013538,14.301567107443,-7.88680176077315));
#66400=CARTESIAN_POINT('Ctrl Pts',(-20.3715787455926,14.3283070841755,-7.75003309890807));
#66401=CARTESIAN_POINT('Ctrl Pts',(-20.3637812898313,14.3482937650472,-7.61233011358183));
#66402=CARTESIAN_POINT('Ctrl Pts',(-20.356172729412,14.3677962635095,-7.47796301797296));
#66403=CARTESIAN_POINT('Ctrl Pts',(-20.3485641689927,14.3808689065492,-7.34270661697724));
#66404=CARTESIAN_POINT('Ctrl Pts',(-20.3409556085734,14.3874635719564,-7.20715988967947));
#66405=CARTESIAN_POINT('Ctrl Pts',(-20.3330637051412,14.3943038228966,-7.06656539828703));
#66406=CARTESIAN_POINT('Ctrl Pts',(-20.325171801709,14.3941742794439,-6.92565884820072));
#66407=CARTESIAN_POINT('Ctrl Pts',(-20.3172798982768,14.3870804471944,-6.78510994516341));
#66408=CARTESIAN_POINT('Ctrl Pts',(-20.3093879948446,14.379986614945,-6.6445610421261));
#66409=CARTESIAN_POINT('Ctrl Pts',(-20.3014960914124,14.3659285138308,-6.50437010302651));
#66410=CARTESIAN_POINT('Ctrl Pts',(-20.2936041879802,14.3449717784631,-6.36520343023823));
#66411=CARTESIAN_POINT('Ctrl Pts',(-20.2865699500337,14.3262925505144,-6.24116092274532));
#66412=CARTESIAN_POINT('Ctrl Pts',(-20.2795357120872,14.3021211905467,-6.11785842915652));
#66413=CARTESIAN_POINT('Ctrl Pts',(-20.2725014741406,14.2725375817417,-5.99580450295988));
#66414=CARTESIAN_POINT('Ctrl Pts',(-20.265471124558,14.2429703260709,-5.87381804534861));
#66415=CARTESIAN_POINT('Ctrl Pts',(-20.2584407749754,14.2079968698656,-5.75307915384293));
#66416=CARTESIAN_POINT('Ctrl Pts',(-20.2514104253928,14.1677481508453,-5.63408606706174));
#66417=CARTESIAN_POINT('Ctrl Pts',(-20.2443818233126,14.1275094362681,-5.51512255785725));
#66418=CARTESIAN_POINT('Ctrl Pts',(-20.2373532212324,14.081998189689,-5.39790435455489));
#66419=CARTESIAN_POINT('Ctrl Pts',(-20.2303246191521,14.0313951170116,-5.2829142433062));
#66420=CARTESIAN_POINT('Ctrl Pts',(-20.2232971566901,13.9808002491211,-5.16794277656471));
#66421=CARTESIAN_POINT('Ctrl Pts',(-20.2162696942281,13.9251153573761,-5.05519903309845));
#66422=CARTESIAN_POINT('Ctrl Pts',(-20.2092422317661,13.864568966409,-4.94514506201334));
#66423=CARTESIAN_POINT('Ctrl Pts',(-20.2022129155991,13.8040066045073,-4.83506206087784));
#66424=CARTESIAN_POINT('Ctrl Pts',(-20.1951835994321,13.7385803675296,-4.72767058650132));
#66425=CARTESIAN_POINT('Ctrl Pts',(-20.1881542832652,13.668564345964,-4.62340736449718));
#66426=CARTESIAN_POINT('Ctrl Pts',(-20.1845223698675,13.6323884049852,-4.5695365492016));
#66427=CARTESIAN_POINT('Ctrl Pts',(-20.1808904564697,13.5949879020393,-4.51650039912015));
#66428=CARTESIAN_POINT('Ctrl Pts',(-20.177258543072,13.556405113779,-4.4643560302843));
#66429=CARTESIAN_POINT('Ctrl Pts',(-20.1698758048977,13.4779763098484,-4.35836004959168));
#66430=CARTESIAN_POINT('Ctrl Pts',(-20.1624930667234,13.3946337929648,-4.25601561199655));
#66431=CARTESIAN_POINT('Ctrl Pts',(-20.1551103285491,13.3067375194271,-4.15775955536042));
#66432=CARTESIAN_POINT('Ctrl Pts',(-20.1477267136224,13.2188308075853,-4.05949183012278));
#66433=CARTESIAN_POINT('Ctrl Pts',(-20.1403430986957,13.1263694729261,-3.96531369053039));
#66434=CARTESIAN_POINT('Ctrl Pts',(-20.132959483769,13.0297520661519,-3.87562695044562));
#66435=CARTESIAN_POINT('Ctrl Pts',(-20.1255738893439,12.9331087568887,-3.78591616593788));
#66436=CARTESIAN_POINT('Ctrl Pts',(-20.1181882949188,12.8323073816896,-3.70069940365669));
#66437=CARTESIAN_POINT('Ctrl Pts',(-20.1108027004937,12.7277819172479,-3.62034024219851));
#66438=CARTESIAN_POINT('Ctrl Pts',(-20.103416930456,12.62325396743,-3.5399791699835));
#66439=CARTESIAN_POINT('Ctrl Pts',(-20.0960311604184,12.5150020057933,-3.46447611991925));
#66440=CARTESIAN_POINT('Ctrl Pts',(-20.0886453903808,12.4034914669734,-3.39415310805738));
#66441=CARTESIAN_POINT('Ctrl Pts',(-20.0812586628136,12.2919664713494,-3.32382097915588));
#66442=CARTESIAN_POINT('Ctrl Pts',(-20.0738719352465,12.1771823237382,-3.25867039897299));
#66443=CARTESIAN_POINT('Ctrl Pts',(-20.0664852076794,12.0596321377066,-3.19897922513017));
#66444=CARTESIAN_POINT('Ctrl Pts',(-20.0646277711742,12.030073445479,-3.18396952505323));
#66445=CARTESIAN_POINT('Ctrl Pts',(-20.062770334669,12.000339980668,-3.16930479834316));
#66446=CARTESIAN_POINT('Ctrl Pts',(-20.0609128981638,11.9704398252603,-3.15498900394674));
#66447=CARTESIAN_POINT('Ctrl Pts',(-20.0537147341779,11.8545671043196,-3.09951069533852));
#66448=CARTESIAN_POINT('Ctrl Pts',(-20.0465165701919,11.7361510511272,-3.04925809080175));
#66449=CARTESIAN_POINT('Ctrl Pts',(-20.039318406206,11.6156836829833,-3.00444909174791));
#66450=CARTESIAN_POINT('Ctrl Pts',(-20.0321223301932,11.495251258838,-2.95965309045125));
#66451=CARTESIAN_POINT('Ctrl Pts',(-20.0249262541804,11.3727690395134,-2.92029767028471));
#66452=CARTESIAN_POINT('Ctrl Pts',(-20.0177301781676,11.2487478957301,-2.88655215811556));
#66453=CARTESIAN_POINT('Ctrl Pts',(-20.0105343327563,11.1247307262596,-2.85280772733637));
#66454=CARTESIAN_POINT('Ctrl Pts',(-20.003338487345,10.9991750728829,-2.82467294395313));
#66455=CARTESIAN_POINT('Ctrl Pts',(-19.9961426419336,10.8726059996031,-2.80226698403128));
#66456=CARTESIAN_POINT('Ctrl Pts',(-19.9889472731621,10.746045310029,-2.77986250823955));
#66457=CARTESIAN_POINT('Ctrl Pts',(-19.9817519043905,10.6184716854824,-2.76318615803964));
#66458=CARTESIAN_POINT('Ctrl Pts',(-19.9745565356189,10.4904191279099,-2.75230575687129));
#66459=CARTESIAN_POINT('Ctrl Pts',(-19.9673594219651,10.3623355174989,-2.74142271719775));
#66460=CARTESIAN_POINT('Ctrl Pts',(-19.9601623083114,10.2337730969215,-2.73633846333066));
#66461=CARTESIAN_POINT('Ctrl Pts',(-19.9529651946576,10.1052700053776,-2.73706885965061));
#66462=CARTESIAN_POINT('Ctrl Pts',(-19.950165880857,10.0552887913946,-2.73735294693847));
#66463=CARTESIAN_POINT('Ctrl Pts',(-19.9473665670563,10.0053165643208,-2.73851612639266));
#66464=CARTESIAN_POINT('Ctrl Pts',(-19.9445672532556,9.95538496385429,-2.74055720144196));
#66465=CARTESIAN_POINT('Ctrl Pts',(-19.9372996658139,9.82575238303743,-2.74585624701248));
#66466=CARTESIAN_POINT('Ctrl Pts',(-19.9300320783721,9.69634259000923,-2.75707830985315));
#66467=CARTESIAN_POINT('Ctrl Pts',(-19.9227644909304,9.56770226521737,-2.77418028008848));
#66468=CARTESIAN_POINT('Ctrl Pts',(-19.9154981270172,9.4390835975591,-2.791279371136));
#66469=CARTESIAN_POINT('Ctrl Pts',(-19.908231763104,9.31123447891631,-2.81425634945049));
#66470=CARTESIAN_POINT('Ctrl Pts',(-19.9009653991908,9.18469503787924,-2.8430164080728));
#66471=CARTESIAN_POINT('Ctrl Pts',(-19.8936986728736,9.05814928578943,-2.87177790107988));
#66472=CARTESIAN_POINT('Ctrl Pts',(-19.8864319465564,8.93291367641405,-2.90632297800972));
#66473=CARTESIAN_POINT('Ctrl Pts',(-19.8791652202392,8.80951708114262,-2.94650594006544));
#66474=CARTESIAN_POINT('Ctrl Pts',(-19.8718988049651,8.68612576770948,-2.98668718213929));
#66475=CARTESIAN_POINT('Ctrl Pts',(-19.8646323896911,8.56457363589267,-3.03250571882476));
#66476=CARTESIAN_POINT('Ctrl Pts',(-19.8573659744171,8.44537320366214,-3.08376635862251));
#66477=CARTESIAN_POINT('Ctrl Pts',(-19.8500981487013,8.32614963412624,-3.1350369483261));
#66478=CARTESIAN_POINT('Ctrl Pts',(-19.8428303229855,8.20927899029798,-3.19175161528081));
#66479=CARTESIAN_POINT('Ctrl Pts',(-19.8355624972697,8.09525300626815,-3.25366737081543));
#66480=CARTESIAN_POINT('Ctrl Pts',(-19.8331155342956,8.05686224513593,-3.27451343499348));
#66481=CARTESIAN_POINT('Ctrl Pts',(-19.8306685713215,8.01879374688149,-3.29594868576314));
#66482=CARTESIAN_POINT('Ctrl Pts',(-19.8282216083474,7.98106564680016,-3.3179626794408));
#66483=CARTESIAN_POINT('Ctrl Pts',(-19.8209722445845,7.8692925123192,-3.38318125844403));
#66484=CARTESIAN_POINT('Ctrl Pts',(-19.8137228808216,7.76047097522316,-3.45350495882227));
#66485=CARTESIAN_POINT('Ctrl Pts',(-19.8064735170587,7.65506214645853,-3.5286420079512));
#66486=CARTESIAN_POINT('Ctrl Pts',(-19.7992255772224,7.54967402219211,-3.60376429859246));
#66487=CARTESIAN_POINT('Ctrl Pts',(-19.7919776373861,7.44769755071203,-3.68369785128094));
#66488=CARTESIAN_POINT('Ctrl Pts',(-19.7847296975498,7.34956393018538,-3.76810822462391));
#66489=CARTESIAN_POINT('Ctrl Pts',(-19.777481498792,7.25142680398565,-3.85252161339799));
#66490=CARTESIAN_POINT('Ctrl Pts',(-19.7702333000342,7.15713306776873,-3.94141191953554));
#66491=CARTESIAN_POINT('Ctrl Pts',(-19.7629851012764,7.06708019444085,-4.03440496113865));
#66492=CARTESIAN_POINT('Ctrl Pts',(-19.7557372208103,6.97703127562475,-4.12739391911772));
#66493=CARTESIAN_POINT('Ctrl Pts',(-19.7484893403443,6.89122308655681,-4.22448500231484));
#66494=CARTESIAN_POINT('Ctrl Pts',(-19.7412414598782,6.81001549954522,-4.32526792907393));
#66495=CARTESIAN_POINT('Ctrl Pts',(-19.7339920212989,6.72879045493104,-4.42607252164463));
#66496=CARTESIAN_POINT('Ctrl Pts',(-19.7267425827196,6.65216820444815,-4.53057027310971));
#66497=CARTESIAN_POINT('Ctrl Pts',(-19.7194931441403,6.58046788328555,-4.63831838840851));
#66498=CARTESIAN_POINT('Ctrl Pts',(-19.7169540839066,6.55535539599213,-4.6760563389847));
#66499=CARTESIAN_POINT('Ctrl Pts',(-19.7144150236729,6.53084629803888,-4.71419274091907));
#66500=CARTESIAN_POINT('Ctrl Pts',(-19.7118759634392,6.50695304158714,-4.7527077328274));
#66501=CARTESIAN_POINT('Ctrl Pts',(-19.7046273272713,6.43874137784321,-4.86266225838396));
#66502=CARTESIAN_POINT('Ctrl Pts',(-19.6973786911033,6.37552683267345,-4.97574519864636));
#66503=CARTESIAN_POINT('Ctrl Pts',(-19.6901300549354,6.31758028923035,-5.09148300540817));
#66504=CARTESIAN_POINT('Ctrl Pts',(-19.6828828888796,6.25964549805596,-5.20719733912528));
#66505=CARTESIAN_POINT('Ctrl Pts',(-19.6756357228238,6.20697673229024,-5.3255651559131));
#66506=CARTESIAN_POINT('Ctrl Pts',(-19.6683885567681,6.15979847242466,-5.44608919755154));
#66507=CARTESIAN_POINT('Ctrl Pts',(-19.6611411920792,6.1126189194791,-5.5666165425595));
#66508=CARTESIAN_POINT('Ctrl Pts',(-19.6538938273903,6.07093030282521,-5.68929990953642));
#66509=CARTESIAN_POINT('Ctrl Pts',(-19.6466464627014,6.03490869934269,-5.81362270732221));
#66510=CARTESIAN_POINT('Ctrl Pts',(-19.6393994491196,5.99888884096896,-5.9379394821444));
#66511=CARTESIAN_POINT('Ctrl Pts',(-19.6321524355377,5.96853554134302,-6.06389519594937));
#66512=CARTESIAN_POINT('Ctrl Pts',(-19.6249054219559,5.94397475426181,-6.19095895203749));
#66513=CARTESIAN_POINT('Ctrl Pts',(-19.6176568912815,5.91940882561603,-6.31804930770098));
#66514=CARTESIAN_POINT('Ctrl Pts',(-19.6104083606071,5.90063789667634,-6.44624782889921));
#66515=CARTESIAN_POINT('Ctrl Pts',(-19.6031598299327,5.88773670376587,-6.575013954675));
#66516=CARTESIAN_POINT('Ctrl Pts',(-19.6006166594655,5.88321027844253,-6.62019196701424));
#66517=CARTESIAN_POINT('Ctrl Pts',(-19.5980734889982,5.87940594047427,-6.66543979058032));
#66518=CARTESIAN_POINT('Ctrl Pts',(-19.595530318531,5.87632540455801,-6.71073392752201));
#66519=CARTESIAN_POINT('Ctrl Pts',(-19.5882769227069,5.86753938465133,-6.8399176798439));
#66520=CARTESIAN_POINT('Ctrl Pts',(-19.5810235268829,5.8646418040146,-6.969524604123));
#66521=CARTESIAN_POINT('Ctrl Pts',(-19.5737701310588,5.86764989988178,-7.09900870730542));
#66522=CARTESIAN_POINT('Ctrl Pts',(-19.56651812171,5.8706574207561,-7.22846805980276));
#66523=CARTESIAN_POINT('Ctrl Pts',(-19.5592661123613,5.87956835819632,-7.35780429308268));
#66524=CARTESIAN_POINT('Ctrl Pts',(-19.5520141030125,5.89434784617514,-7.48647223348577));
#66525=CARTESIAN_POINT('Ctrl Pts',(-19.5447618211018,5.90912788963121,-7.61514500978809));
#66526=CARTESIAN_POINT('Ctrl Pts',(-19.5375095391911,5.9297768885282,-7.74314909965177));
#66527=CARTESIAN_POINT('Ctrl Pts',(-19.5302572572804,5.95620815783502,-7.869944940855));
#66528=CARTESIAN_POINT('Ctrl Pts',(-19.5230052970079,5.98263825491685,-7.99673515867135));
#66529=CARTESIAN_POINT('Ctrl Pts',(-19.5157533367354,6.01485003720225,-8.12231689743408));
#66530=CARTESIAN_POINT('Ctrl Pts',(-19.5085013764629,6.05270583759639,-8.24616144916773));
#66531=CARTESIAN_POINT('Ctrl Pts',(-19.5012478974044,6.09056956617225,-8.37003193780146));
#66532=CARTESIAN_POINT('Ctrl Pts',(-19.4939944183459,6.13407957230502,-8.49216418269563));
#66533=CARTESIAN_POINT('Ctrl Pts',(-19.4867409392874,6.18304841315165,-8.61204493506296));
#66534=CARTESIAN_POINT('Ctrl Pts',(-19.4842221840659,6.20005273929354,-8.65367327210638));
#66535=CARTESIAN_POINT('Ctrl Pts',(-19.4817034288444,6.21771486629463,-8.69503028409148));
#66536=CARTESIAN_POINT('Ctrl Pts',(-19.4791846736229,6.23602558437293,-8.73609503624007));
#66537=CARTESIAN_POINT('Ctrl Pts',(-19.4719351321326,6.28872793086994,-8.8542885875413));
#66538=CARTESIAN_POINT('Ctrl Pts',(-19.4646855906423,6.34682588834277,-8.97010224507851));
#66539=CARTESIAN_POINT('Ctrl Pts',(-19.4574360491521,6.41007951261352,-9.08304590396125));
#66540=CARTESIAN_POINT('Ctrl Pts',(-19.4501879543185,6.4733205145299,-9.19596702476964));
#66541=CARTESIAN_POINT('Ctrl Pts',(-19.442939859485,6.54171496200513,-9.30601898763982));
#66542=CARTESIAN_POINT('Ctrl Pts',(-19.4356917646515,6.61497724357959,-9.41273678518878));
#66543=CARTESIAN_POINT('Ctrl Pts',(-19.4284434460103,6.6882417873569,-9.51945787798464));
#66544=CARTESIAN_POINT('Ctrl Pts',(-19.421195127369,6.76637427283083,-9.62284431239772));
#66545=CARTESIAN_POINT('Ctrl Pts',(-19.4139468087278,6.84904591912196,-9.7224602886453));
#66546=CARTESIAN_POINT('Ctrl Pts',(-19.4066988291477,6.93171369820757,-9.82207160506727));
#66547=CARTESIAN_POINT('Ctrl Pts',(-19.3994508495676,7.01891999109499,-9.91791255098534));
#66548=CARTESIAN_POINT('Ctrl Pts',(-19.3922028699875,7.11029604323606,-10.0095807793547));
#66549=CARTESIAN_POINT('Ctrl Pts',(-19.384953363692,7.20169134284058,-10.1012683167315));
#66550=CARTESIAN_POINT('Ctrl Pts',(-19.3777038573965,7.29725791129566,-10.1887811363229));
#66551=CARTESIAN_POINT('Ctrl Pts',(-19.370454351101,7.39659024575933,-10.2717538530849));
#66552=CARTESIAN_POINT('Ctrl Pts',(-19.3679159103056,7.43137182119772,-10.3008070493374));
#66553=CARTESIAN_POINT('Ctrl Pts',(-19.3653774695102,7.46661479837169,-10.3293039451163));
#66554=CARTESIAN_POINT('Ctrl Pts',(-19.3628390287147,7.50230080009072,-10.3572300135671));
#66555=CARTESIAN_POINT('Ctrl Pts',(-19.3555873220309,7.60424700961119,-10.4370079849911));
#66556=CARTESIAN_POINT('Ctrl Pts',(-19.348335615347,7.70984795365347,-10.5121532289869));
#66557=CARTESIAN_POINT('Ctrl Pts',(-19.3410839086632,7.81866176481192,-10.5823449932681));
#66558=CARTESIAN_POINT('Ctrl Pts',(-19.3338336170501,7.92745434245319,-10.6525230605928));
#66559=CARTESIAN_POINT('Ctrl Pts',(-19.3265833254369,8.03945824632693,-10.7177493891838));
#66560=CARTESIAN_POINT('Ctrl Pts',(-19.3193330338238,8.15420302405171,-10.7777467962808));
#66561=CARTESIAN_POINT('Ctrl Pts',(-19.312082494214,8.26895172662819,-10.8377462555925));
#66562=CARTESIAN_POINT('Ctrl Pts',(-19.3048319546043,8.38644118586107,-10.8925162726726));
#66563=CARTESIAN_POINT('Ctrl Pts',(-19.2975814149945,8.5061764926047,-10.9418256925361));
#66564=CARTESIAN_POINT('Ctrl Pts',(-19.290331206482,8.62590633161308,-10.9911328606757));
#66565=CARTESIAN_POINT('Ctrl Pts',(-19.2830809979695,8.74788149278864,-11.0349798004483));
#66566=CARTESIAN_POINT('Ctrl Pts',(-19.2758307894569,8.87158741976644,-11.0731836369712));
#66567=CARTESIAN_POINT('Ctrl Pts',(-19.2685790612726,8.99531927598627,-11.1113954811665));
#66568=CARTESIAN_POINT('Ctrl Pts',(-19.2613273330882,9.12078229219613,-11.143961758176));
#66569=CARTESIAN_POINT('Ctrl Pts',(-19.2540756049039,9.24744675522654,-11.1707494618335));
#66570=CARTESIAN_POINT('Ctrl Pts',(-19.2515481978714,9.29159246042793,-11.180085640588));
#66571=CARTESIAN_POINT('Ctrl Pts',(-19.249020790839,9.33588399625009,-11.1887203497344));
#66572=CARTESIAN_POINT('Ctrl Pts',(-19.2464933838065,9.38029862923168,-11.1966494142398));
#66573=CARTESIAN_POINT('Ctrl Pts',(-19.239033624303,9.51139048591435,-11.220052417214));
#66574=CARTESIAN_POINT('Ctrl Pts',(-19.2315738647995,9.64359095899357,-11.2373107330629));
#66575=CARTESIAN_POINT('Ctrl Pts',(-19.224114105296,9.77632784658091,-11.2483453755609));
#66576=CARTESIAN_POINT('Ctrl Pts',(-19.2175155133523,9.8937413579231,-11.2581061598134));
#66577=CARTESIAN_POINT('Ctrl Pts',(-19.2109169214085,10.0115743103388,-11.2629979844182));
#66578=CARTESIAN_POINT('Ctrl Pts',(-19.2043183294647,10.1294271144268,-11.2629999993769));
#66579=CARTESIAN_POINT('Ctrl Pts',(-19.2043183294109,10.1294271153884,-11.2629999993769));
#66580=CARTESIAN_POINT('Ctrl Pts',(-19.1970583198552,10.2590930336831,-11.2630022162782));
#66581=CARTESIAN_POINT('Ctrl Pts',(-19.1897983102996,10.3887626081957,-11.257084097175));
#66582=CARTESIAN_POINT('Ctrl Pts',(-19.182538300744,10.5178887238751,-11.2452706862068));
#66583=CARTESIAN_POINT('Ctrl Pts',(-19.175278526011,10.6470106630119,-11.2334576573395));
#66584=CARTESIAN_POINT('Ctrl Pts',(-19.168018751278,10.7755888364936,-11.2157497517238));
#66585=CARTESIAN_POINT('Ctrl Pts',(-19.160758976545,10.9030811422902,-11.1922238986358));
#66586=CARTESIAN_POINT('Ctrl Pts',(-19.1534975321505,11.0306027697949,-11.1686926348825));
#66587=CARTESIAN_POINT('Ctrl Pts',(-19.1462360877561,11.1570376928693,-11.1393408138078));
#66588=CARTESIAN_POINT('Ctrl Pts',(-19.1389746433616,11.2818534964405,-11.1042965803218));
#66589=CARTESIAN_POINT('Ctrl Pts',(-19.1360323418738,11.3324282450154,-11.0900968295944));
#66590=CARTESIAN_POINT('Ctrl Pts',(-19.1330900403861,11.3827373049399,-11.0749630604004));
#66591=CARTESIAN_POINT('Ctrl Pts',(-19.1301477388984,11.4327459192928,-11.0589061425274));
#66592=CARTESIAN_POINT('Ctrl Pts',(-19.1264842467592,11.4950121983722,-11.0389134964128));
#66593=CARTESIAN_POINT('Ctrl Pts',(-19.1228207546201,11.5568240284571,-11.0174859462435));
#66594=CARTESIAN_POINT('Ctrl Pts',(-19.1191572624809,11.6181146495903,-10.9946458447559));
#66595=CARTESIAN_POINT('',(-19.613681670589,10.1296816520865,-11.2629999961298));
#66596=CARTESIAN_POINT('Ctrl Pts',(-19.5287463281039,11.618114650837,-10.9946458442913));
#66597=CARTESIAN_POINT('Ctrl Pts',(-19.5427543530944,11.3829167082039,-11.0822929391522));
#66598=CARTESIAN_POINT('Ctrl Pts',(-19.5565651777506,11.1404319869351,-11.1489989699717));
#66599=CARTESIAN_POINT('Ctrl Pts',(-19.584788886185,10.641461197615,-11.2398924321116));
#66600=CARTESIAN_POINT('Ctrl Pts',(-19.5992884130183,10.3858268071179,-11.2629888708551));
#66601=CARTESIAN_POINT('Ctrl Pts',(-19.6137437660346,10.1296851569352,-11.262999995979));
#66602=CARTESIAN_POINT('Ctrl Pts',(-19.613681670589,10.1296816520865,-11.2629999961298));
#66603=CARTESIAN_POINT('Ctrl Pts',(-19.6210625559268,9.99792696780947,-11.2630056103717));
#66604=CARTESIAN_POINT('Ctrl Pts',(-19.6284434412646,9.86616452721088,-11.2568987546168));
#66605=CARTESIAN_POINT('Ctrl Pts',(-19.6358243266025,9.73495915245449,-11.2447033488358));
#66606=CARTESIAN_POINT('Ctrl Pts',(-19.6432038414137,9.60377814069074,-11.2325102075702));
#66607=CARTESIAN_POINT('Ctrl Pts',(-19.6505833562249,9.47315430553389,-11.2142308037361));
#66608=CARTESIAN_POINT('Ctrl Pts',(-19.6579628710361,9.34364777489142,-11.1899409638194));
#66609=CARTESIAN_POINT('Ctrl Pts',(-19.665341452104,9.21415763094539,-11.1656541973403));
#66610=CARTESIAN_POINT('Ctrl Pts',(-19.6727200331718,9.0857848227637,-11.1353585705236));
#66611=CARTESIAN_POINT('Ctrl Pts',(-19.6800986142396,8.95908014795422,-11.0991811828629));
#66612=CARTESIAN_POINT('Ctrl Pts',(-19.6849303155029,8.87611038293851,-11.0754912175352));
#66613=CARTESIAN_POINT('Ctrl Pts',(-19.6897620167663,8.79385571635695,-11.049280203234));
#66614=CARTESIAN_POINT('Ctrl Pts',(-19.6945937180296,8.71246771439215,-11.0205955406563));
#66615=CARTESIAN_POINT('Ctrl Pts',(-19.7016228891401,8.59406424510147,-10.9788650216284));
#66616=CARTESIAN_POINT('Ctrl Pts',(-19.7086520602506,8.47745739883753,-10.9318830738138));
#66617=CARTESIAN_POINT('Ctrl Pts',(-19.7156812313611,8.36312882780601,-10.8798327131517));
#66618=CARTESIAN_POINT('Ctrl Pts',(-19.7227086284805,8.24882911051486,-10.82779548873));
#66619=CARTESIAN_POINT('Ctrl Pts',(-19.7297360255998,8.13680687283187,-10.7706925591275));
#66620=CARTESIAN_POINT('Ctrl Pts',(-19.7367634227191,8.02752294555477,-10.7087547050979));
#66621=CARTESIAN_POINT('Ctrl Pts',(-19.7437922455919,7.91821684620777,-10.6468042848066));
#66622=CARTESIAN_POINT('Ctrl Pts',(-19.7508210684647,7.8116505045704,-10.5800171656424));
#66623=CARTESIAN_POINT('Ctrl Pts',(-19.7578498913375,7.70825937959702,-10.5086696707029));
#66624=CARTESIAN_POINT('Ctrl Pts',(-19.7648793838462,7.60485840455196,-10.4373153784882));
#66625=CARTESIAN_POINT('Ctrl Pts',(-19.7719088763549,7.50463356199163,-10.3614000686881));
#66626=CARTESIAN_POINT('Ctrl Pts',(-19.7789383688636,7.40798992434636,-10.2812424336089));
#66627=CARTESIAN_POINT('Ctrl Pts',(-19.7859724420486,7.31128331014651,-10.2010325648618));
#66628=CARTESIAN_POINT('Ctrl Pts',(-19.7930065152336,7.21816285464981,-10.1165750994141));
#66629=CARTESIAN_POINT('Ctrl Pts',(-19.8000405884186,7.12899939384763,-10.0282280482948));
#66630=CARTESIAN_POINT('Ctrl Pts',(-19.8036735132583,7.08294867145319,-9.98259898131086));
#66631=CARTESIAN_POINT('Ctrl Pts',(-19.807306438098,7.03795286658765,-9.93593298706528));
#66632=CARTESIAN_POINT('Ctrl Pts',(-19.8109393629378,6.99405904894667,-9.88828306134593));
#66633=CARTESIAN_POINT('Ctrl Pts',(-19.8185514682813,6.90208787460305,-9.78844167453286));
#66634=CARTESIAN_POINT('Ctrl Pts',(-19.8261635736248,6.81489782850554,-9.68421427120516));
#66635=CARTESIAN_POINT('Ctrl Pts',(-19.8337756789683,6.73287352582023,-9.57606242061428));
#66636=CARTESIAN_POINT('Ctrl Pts',(-19.8415681230414,6.64890598169537,-9.46534833967273));
#66637=CARTESIAN_POINT('Ctrl Pts',(-19.8493605671145,6.5703521935622,-9.35052175498863));
#66638=CARTESIAN_POINT('Ctrl Pts',(-19.8571530111877,6.49757984993105,-9.23211223363054));
#66639=CARTESIAN_POINT('Ctrl Pts',(-19.8647591278018,6.42654758755655,-9.11653403772446));
#66640=CARTESIAN_POINT('Ctrl Pts',(-19.872365244416,6.36102356679838,-8.99754254531327));
#66641=CARTESIAN_POINT('Ctrl Pts',(-19.8799713610301,6.30130558280906,-8.8756589519921));
#66642=CARTESIAN_POINT('Ctrl Pts',(-19.8878569688327,6.23939322668899,-8.74929667498954));
#66643=CARTESIAN_POINT('Ctrl Pts',(-19.8957425766354,6.18372190273754,-8.61982593912762));
#66644=CARTESIAN_POINT('Ctrl Pts',(-19.903628184438,6.13457147332775,-8.48785586223272));
#66645=CARTESIAN_POINT('Ctrl Pts',(-19.9115137922407,6.08542104391795,-8.35588578533781));
#66646=CARTESIAN_POINT('Ctrl Pts',(-19.9193994000433,6.04279165902778,-8.22141665147341));
#66647=CARTESIAN_POINT('Ctrl Pts',(-19.927285007846,6.00690792403289,-8.085082289586));
#66648=CARTESIAN_POINT('Ctrl Pts',(-19.9343237861388,5.97487771643589,-7.96338877260736));
#66649=CARTESIAN_POINT('Ctrl Pts',(-19.9413625644316,5.94823387545845,-7.8402524200153));
#66650=CARTESIAN_POINT('Ctrl Pts',(-19.9484013427244,5.92708903886797,-7.71617812990721));
#66651=CARTESIAN_POINT('Ctrl Pts',(-19.9554399109056,5.90594483346336,-7.59210754349001));
#66652=CARTESIAN_POINT('Ctrl Pts',(-19.9624784790867,5.89029936842274,-7.46709945251523));
#66653=CARTESIAN_POINT('Ctrl Pts',(-19.9695170472678,5.8802139040895,-7.3416674920177));
#66654=CARTESIAN_POINT('Ctrl Pts',(-19.9765593081639,5.87012314851751,-7.21616972488726));
#66655=CARTESIAN_POINT('Ctrl Pts',(-19.9836015690599,5.86559825316507,-7.0902480255059));
#66656=CARTESIAN_POINT('Ctrl Pts',(-19.990643829956,5.86664848269717,-6.96441992932841));
#66657=CARTESIAN_POINT('Ctrl Pts',(-19.9976880482936,5.86769900414732,-6.83855685842447));
#66658=CARTESIAN_POINT('Ctrl Pts',(-20.0047322666312,5.87432772657293,-6.71278782503369));
#66659=CARTESIAN_POINT('Ctrl Pts',(-20.0117764849689,5.88649181534104,-6.58762814727832));
#66660=CARTESIAN_POINT('Ctrl Pts',(-20.0188271374083,5.89866701463715,-6.46235415022382));
#66661=CARTESIAN_POINT('Ctrl Pts',(-20.0258777898477,5.91638763336263,-6.33769100055036));
#66662=CARTESIAN_POINT('Ctrl Pts',(-20.0329284422871,5.93955916974701,-6.21414706275352));
#66663=CARTESIAN_POINT('Ctrl Pts',(-20.0364958457761,5.95128322230163,-6.15163780158474));
#66664=CARTESIAN_POINT('Ctrl Pts',(-20.0400632492651,5.96440191628728,-6.08941489423676));
#66665=CARTESIAN_POINT('Ctrl Pts',(-20.0436306527542,5.97889809135828,-6.02754290789789));
#66666=CARTESIAN_POINT('Ctrl Pts',(-20.0506540818166,6.00743785637264,-5.90573064070087));
#66667=CARTESIAN_POINT('Ctrl Pts',(-20.0576775108791,6.04137122992328,-5.78506070393765));
#66668=CARTESIAN_POINT('Ctrl Pts',(-20.0647009399416,6.08058632073389,-5.6660333520467));
#66669=CARTESIAN_POINT('Ctrl Pts',(-20.0717185423857,6.11976887880798,-5.54710474493479));
#66670=CARTESIAN_POINT('Ctrl Pts',(-20.0787361448298,6.16422430917893,-5.42981637531585));
#66671=CARTESIAN_POINT('Ctrl Pts',(-20.085753747274,6.21379041548669,-5.3146550947208));
#66672=CARTESIAN_POINT('Ctrl Pts',(-20.0927670920274,6.2633264492517,-5.19956368430097));
#66673=CARTESIAN_POINT('Ctrl Pts',(-20.0997804367809,6.31796683139565,-5.08659714716067));
#66674=CARTESIAN_POINT('Ctrl Pts',(-20.1067937815343,6.37750071407498,-4.97622373805349));
#66675=CARTESIAN_POINT('Ctrl Pts',(-20.1138574549108,6.43746181920613,-4.86505827581068));
#66676=CARTESIAN_POINT('Ctrl Pts',(-20.1209211282873,6.5023867959048,-4.75652367863071));
#66677=CARTESIAN_POINT('Ctrl Pts',(-20.1279848016638,6.57201228474143,-4.65107468067111));
#66678=CARTESIAN_POINT('Ctrl Pts',(-20.1349957589147,6.64111815923273,-4.54641264755664));
#66679=CARTESIAN_POINT('Ctrl Pts',(-20.1420067161656,6.71485438329882,-4.44479062478944));
#66680=CARTESIAN_POINT('Ctrl Pts',(-20.1490176734164,6.79291940437145,-4.34662499279219));
#66681=CARTESIAN_POINT('Ctrl Pts',(-20.1560293038896,6.87099192158304,-4.2484499345089));
#66682=CARTESIAN_POINT('Ctrl Pts',(-20.1630409343627,6.95339382288946,-4.15373223076921));
#66683=CARTESIAN_POINT('Ctrl Pts',(-20.1700525648358,7.03978297499938,-4.06285551846333));
#66684=CARTESIAN_POINT('Ctrl Pts',(-20.1770662859279,7.12619788528295,-3.97195170995291));
#66685=CARTESIAN_POINT('Ctrl Pts',(-20.1840800070199,7.21660214710082,-3.88489145349599));
#66686=CARTESIAN_POINT('Ctrl Pts',(-20.191093728112,7.3106167200912,-3.80202156757576));
#66687=CARTESIAN_POINT('Ctrl Pts',(-20.1981960793168,7.4058193246704,-3.71810448185337));
#66688=CARTESIAN_POINT('Ctrl Pts',(-20.2052984305217,7.50472380869981,-3.63848467191371));
#66689=CARTESIAN_POINT('Ctrl Pts',(-20.2124007817266,7.6069029600472,-3.5634794960569));
#66690=CARTESIAN_POINT('Ctrl Pts',(-20.2194267016631,7.70798252029948,-3.4892814811754));
#66691=CARTESIAN_POINT('Ctrl Pts',(-20.2264526215996,7.81226625486711,-3.41959943125368));
#66692=CARTESIAN_POINT('Ctrl Pts',(-20.2334785415361,7.91931293289363,-3.3546958798482));
#66693=CARTESIAN_POINT('Ctrl Pts',(-20.2406191083752,8.02810636724196,-3.28873325131098));
#66694=CARTESIAN_POINT('Ctrl Pts',(-20.2477596752143,8.13975333669771,-3.22770663540868));
#66695=CARTESIAN_POINT('Ctrl Pts',(-20.2549002420533,8.25376708692567,-3.17184182160537));
#66696=CARTESIAN_POINT('Ctrl Pts',(-20.2620408088924,8.36778083715362,-3.11597700780207));
#66697=CARTESIAN_POINT('Ctrl Pts',(-20.2691813757315,8.48416096703565,-3.06527411157802));
#66698=CARTESIAN_POINT('Ctrl Pts',(-20.2763219425705,8.60240284429547,-3.0199066245829));
#66699=CARTESIAN_POINT('Ctrl Pts',(-20.2831124685135,8.71484833401245,-2.97676311730259));
#66700=CARTESIAN_POINT('Ctrl Pts',(-20.2899029944564,8.82935140599041,-2.93830145149597));
#66701=CARTESIAN_POINT('Ctrl Pts',(-20.2966935203994,8.94547734886698,-2.90472719326246));
#66702=CARTESIAN_POINT('Ctrl Pts',(-20.3034748353439,9.06144577288687,-2.87119847677993));
#66703=CARTESIAN_POINT('Ctrl Pts',(-20.3102561502883,9.17903229471747,-2.842544107233));
#66704=CARTESIAN_POINT('Ctrl Pts',(-20.3170374652328,9.29778142242843,-2.81892200410919));
#66705=CARTESIAN_POINT('Ctrl Pts',(-20.3238114588109,9.41640234404969,-2.79532540430932));
#66706=CARTESIAN_POINT('Ctrl Pts',(-20.330585452389,9.53618296819803,-2.77675035206636));
#66707=CARTESIAN_POINT('Ctrl Pts',(-20.3373594459671,9.65665251765119,-2.76330503122583));
#66708=CARTESIAN_POINT('Ctrl Pts',(-20.3441279982186,9.77702529787156,-2.74987051056998));
#66709=CARTESIAN_POINT('Ctrl Pts',(-20.3508965504701,9.89808548802565,-2.74155757451038));
#66710=CARTESIAN_POINT('Ctrl Pts',(-20.3576651027216,10.0193527277818,-2.73842322861328));
#66711=CARTESIAN_POINT('Ctrl Pts',(-20.3644308259848,10.1405692826068,-2.73529019274934));
#66712=CARTESIAN_POINT('Ctrl Pts',(-20.371196549248,10.2619922966189,-2.73733145918129));
#66713=CARTESIAN_POINT('Ctrl Pts',(-20.3779622725112,10.383137499644,-2.74455207777438));
#66714=CARTESIAN_POINT('Ctrl Pts',(-20.384726762254,10.5042606155877,-2.75177137991097));
#66715=CARTESIAN_POINT('Ctrl Pts',(-20.3914912519967,10.6251056025061,-2.7641681330934));
#66716=CARTESIAN_POINT('Ctrl Pts',(-20.3982557417395,10.7451902242561,-2.78169529932278));
#66717=CARTESIAN_POINT('Ctrl Pts',(-20.405020688733,10.8652829632157,-2.79922365031404));
#66718=CARTESIAN_POINT('Ctrl Pts',(-20.4117856357265,10.9846148196652,-2.82188304272845));
#66719=CARTESIAN_POINT('Ctrl Pts',(-20.41855058272,11.1027114907248,-2.84957491402132));
#66720=CARTESIAN_POINT('Ctrl Pts',(-20.4253176780028,11.2208456647849,-2.87727557919678));
#66721=CARTESIAN_POINT('Ctrl Pts',(-20.4320847732856,11.3377434657248,-2.91001180325871));
#66722=CARTESIAN_POINT('Ctrl Pts',(-20.4388518685683,11.4529443165418,-2.9476347473342));
#66723=CARTESIAN_POINT('Ctrl Pts',(-20.4456269530807,11.5682811734314,-2.98530210904052));
#66724=CARTESIAN_POINT('Ctrl Pts',(-20.4524020375931,11.6819166829018,-3.0278675742583));
#66725=CARTESIAN_POINT('Ctrl Pts',(-20.4591771221056,11.7934087946616,-3.07513356621555));
#66726=CARTESIAN_POINT('Ctrl Pts',(-20.4659567627322,11.9049758827261,-3.12243134364499));
#66727=CARTESIAN_POINT('Ctrl Pts',(-20.4727364033589,12.0143963278875,-3.1744357569713));
#66728=CARTESIAN_POINT('Ctrl Pts',(-20.4795160439856,12.1212529943158,-3.23090342261781));
#66729=CARTESIAN_POINT('Ctrl Pts',(-20.4863065022887,12.2282801625317,-3.28746118875372));
#66730=CARTESIAN_POINT('Ctrl Pts',(-20.4930969605919,12.3327350284989,-3.34849620756881));
#66731=CARTESIAN_POINT('Ctrl Pts',(-20.499887418895,12.434229583985,-3.41372190917881));
#66732=CARTESIAN_POINT('Ctrl Pts',(-20.5029293567257,12.479696342509,-3.44294122257403));
#66733=CARTESIAN_POINT('Ctrl Pts',(-20.5059712945563,12.5245694743666,-3.47300098129164));
#66734=CARTESIAN_POINT('Ctrl Pts',(-20.5090132323869,12.5688163807365,-3.50387291497142));
#66735=CARTESIAN_POINT('Ctrl Pts',(-20.5160528500654,12.6712120645548,-3.57531639021697));
#66736=CARTESIAN_POINT('Ctrl Pts',(-20.5230924677439,12.7706045269319,-3.65135814019731));
#66737=CARTESIAN_POINT('Ctrl Pts',(-20.5301320854224,12.8665642076717,-3.73172086212295));
#66738=CARTESIAN_POINT('Ctrl Pts',(-20.5371627173815,12.9624014006857,-3.81198100505939));
#66739=CARTESIAN_POINT('Ctrl Pts',(-20.5441933493406,13.0548142404394,-3.89655089391907));
#66740=CARTESIAN_POINT('Ctrl Pts',(-20.5512239812998,13.1434028817285,-3.98511054605499));
#66741=CARTESIAN_POINT('Ctrl Pts',(-20.5582472086855,13.2318982225716,-4.07357692827592));
#66742=CARTESIAN_POINT('Ctrl Pts',(-20.5652704360712,13.3165771118334,-4.16602443564554));
#66743=CARTESIAN_POINT('Ctrl Pts',(-20.5722936634569,13.3970737490667,-4.26209372066711));
#66744=CARTESIAN_POINT('Ctrl Pts',(-20.579352449238,13.477977938426,-4.35864940167621));
#66745=CARTESIAN_POINT('Ctrl Pts',(-20.5864112350191,13.5546571020791,-4.45886338581479));
#66746=CARTESIAN_POINT('Ctrl Pts',(-20.5934700208002,13.6267777203579,-4.56233358584726));
#66747=CARTESIAN_POINT('Ctrl Pts',(-20.6004831025417,13.6984313739637,-4.6651338397634));
#66748=CARTESIAN_POINT('Ctrl Pts',(-20.6074961842832,13.7655851192017,-4.77114794331499));
#66749=CARTESIAN_POINT('Ctrl Pts',(-20.6145092660247,13.8279529364795,-4.87994932215142));
#66750=CARTESIAN_POINT('Ctrl Pts',(-20.6215201005457,13.8903007690717,-4.98871583747262));
#66751=CARTESIAN_POINT('Ctrl Pts',(-20.6285309350668,13.947865534977,-5.10026751473464));
#66752=CARTESIAN_POINT('Ctrl Pts',(-20.6355417695879,14.000405778642,-5.214150775436));
#66753=CARTESIAN_POINT('Ctrl Pts',(-20.6425517747268,14.0529398067936,-5.32802056374194));
#66754=CARTESIAN_POINT('Ctrl Pts',(-20.6495617798658,14.1004503352034,-5.44422103493076));
#66755=CARTESIAN_POINT('Ctrl Pts',(-20.6565717850048,14.1427430711648,-5.56227643416836));
#66756=CARTESIAN_POINT('Ctrl Pts',(-20.6636661797713,14.1855449463016,-5.68175303795214));
#66757=CARTESIAN_POINT('Ctrl Pts',(-20.6707605745379,14.2230024133749,-5.80312915290586));
#66758=CARTESIAN_POINT('Ctrl Pts',(-20.6778549693044,14.2549654534142,-5.92589395649855));
#66759=CARTESIAN_POINT('Ctrl Pts',(-20.6848700180614,14.2865710084581,-6.04728571875378));
#66760=CARTESIAN_POINT('Ctrl Pts',(-20.6918850668184,14.3128043681359,-6.17003487300886));
#66761=CARTESIAN_POINT('Ctrl Pts',(-20.6989001155754,14.3335717231044,-6.29363610865666));
#66762=CARTESIAN_POINT('Ctrl Pts',(-20.7060341833467,14.3546914220416,-6.41933439277077));
#66763=CARTESIAN_POINT('Ctrl Pts',(-20.713168251118,14.37015788043,-6.5459135246403));
#66764=CARTESIAN_POINT('Ctrl Pts',(-20.7203023188893,14.3799273655978,-6.6728361117461));
#66765=CARTESIAN_POINT('Ctrl Pts',(-20.7274363866606,14.3896968507655,-6.79975869885191));
#66766=CARTESIAN_POINT('Ctrl Pts',(-20.7345704544319,14.3937693782952,-6.92702432229997));
#66767=CARTESIAN_POINT('Ctrl Pts',(-20.7417045222032,14.3921567579672,-7.05409587559758));
#66768=CARTESIAN_POINT('Ctrl Pts',(-20.7487553738306,14.3905629482322,-7.17968518832687));
#66769=CARTESIAN_POINT('Ctrl Pts',(-20.755806225458,14.3834131442202,-7.30531135250305));
#66770=CARTESIAN_POINT('Ctrl Pts',(-20.7628570770854,14.3707114727388,-7.43045817858265));
#66771=CARTESIAN_POINT('Ctrl Pts',(-20.7699025977755,14.35801940461,-7.55551038490363));
#66772=CARTESIAN_POINT('Ctrl Pts',(-20.7769481184657,14.339783866004,-7.68008359541989));
#66773=CARTESIAN_POINT('Ctrl Pts',(-20.7839936391558,14.316060990687,-7.80366415327441));
#66774=CARTESIAN_POINT('Ctrl Pts',(-20.7910351758234,14.2923515299169,-7.92717483017315));
#66775=CARTESIAN_POINT('Ctrl Pts',(-20.7980767124911,14.2631609851212,-8.0496935975355));
#66776=CARTESIAN_POINT('Ctrl Pts',(-20.8051182491587,14.2285969725616,-8.17071474302503));
#66777=CARTESIAN_POINT('Ctrl Pts',(-20.8121573620581,14.1940448572855,-8.29169423180984));
#66778=CARTESIAN_POINT('Ctrl Pts',(-20.8191964749575,14.1541230641496,-8.41117675831594));
#66779=CARTESIAN_POINT('Ctrl Pts',(-20.8262355878569,14.108989607831,-8.52866983392907));
#66780=CARTESIAN_POINT('Ctrl Pts',(-20.8332745473014,14.0638571354359,-8.64616034815655));
#66781=CARTESIAN_POINT('Ctrl Pts',(-20.8403135067459,14.0135133592023,-8.76166113931436));
#66782=CARTESIAN_POINT('Ctrl Pts',(-20.8473524661904,13.9581651263394,-8.87469793576249));
#66783=CARTESIAN_POINT('Ctrl Pts',(-20.8509183664974,13.9301259989493,-8.93196178993535));
#66784=CARTESIAN_POINT('Ctrl Pts',(-20.8544842668044,13.9008033009508,-8.98859361159937));
#66785=CARTESIAN_POINT('Ctrl Pts',(-20.8580501671115,13.8702285225073,-9.04453396178702));
#66786=CARTESIAN_POINT('Ctrl Pts',(-20.8656423239006,13.8051317750523,-9.16363653698444));
#66787=CARTESIAN_POINT('Ctrl Pts',(-20.8732344806897,13.7343815652685,-9.27955752070515));
#66788=CARTESIAN_POINT('Ctrl Pts',(-20.8808266374789,13.6583076665164,-9.39179544542065));
#66789=CARTESIAN_POINT('Ctrl Pts',(-20.8886240686906,13.580176904863,-9.50706802495553));
#66790=CARTESIAN_POINT('Ctrl Pts',(-20.8964214999023,13.4964306780399,-9.61845531819866));
#66791=CARTESIAN_POINT('Ctrl Pts',(-20.9042189311141,13.4074713236086,-9.72544913759181));
#66792=CARTESIAN_POINT('Ctrl Pts',(-20.9118275959575,13.3206655674336,-9.82985276616849));
#66793=CARTESIAN_POINT('Ctrl Pts',(-20.9194362608009,13.2288963926098,-9.93007301888365));
#66794=CARTESIAN_POINT('Ctrl Pts',(-20.9270449256444,13.1325767406687,-10.0256733283113));
#66795=CARTESIAN_POINT('Ctrl Pts',(-20.9349367400403,13.032672640352,-10.1248313164362));
#66796=CARTESIAN_POINT('Ctrl Pts',(-20.9428285544361,12.9278730596352,-10.2190186506558));
#66797=CARTESIAN_POINT('Ctrl Pts',(-20.950720368832,12.818679347433,-10.3077913231248));
#66798=CARTESIAN_POINT('Ctrl Pts',(-20.9586121832279,12.7094856352308,-10.3965639955938));
#66799=CARTESIAN_POINT('Ctrl Pts',(-20.9665039976238,12.5958980403164,-10.4799218091269));
#66800=CARTESIAN_POINT('Ctrl Pts',(-20.9743958120197,12.4784556130269,-10.5574677128583));
#66801=CARTESIAN_POINT('Ctrl Pts',(-20.9814300607243,12.3737750920986,-10.6265870744537));
#66802=CARTESIAN_POINT('Ctrl Pts',(-20.9884643094289,12.2659695289948,-10.6911298205444));
#66803=CARTESIAN_POINT('Ctrl Pts',(-20.9954985581336,12.1554703093618,-10.7508150188439));
#66804=CARTESIAN_POINT('Ctrl Pts',(-21.0025288485313,12.045033269762,-10.8104666311358));
#66805=CARTESIAN_POINT('Ctrl Pts',(-21.0095591389291,11.9319059302526,-10.8652659569974));
#66806=CARTESIAN_POINT('Ctrl Pts',(-21.0165894293269,11.8165461611719,-10.9149769156504));
#66807=CARTESIAN_POINT('Ctrl Pts',(-21.0205783820181,11.7510915874208,-10.9431826726081));
#66808=CARTESIAN_POINT('Ctrl Pts',(-21.0245673347093,11.684918780429,-10.969751120246));
#66809=CARTESIAN_POINT('Ctrl Pts',(-21.0285562874006,11.6181146495903,-10.9946458447559));
#66810=CARTESIAN_POINT('Origin',(-23.734,10.1295,-7.));
#66811=CARTESIAN_POINT('',(-22.5286570444943,11.618114651272,-10.9946458441291));
#66812=CARTESIAN_POINT('',(-22.1191569086782,11.6181146495903,-10.9946458447559));
#66813=CARTESIAN_POINT('',(-23.734,11.6181146495903,-10.9946458447559));
#66814=CARTESIAN_POINT('',(-23.534,12.9193325810254,-3.77664721604209));
#66815=CARTESIAN_POINT('Ctrl Pts',(-23.534,12.9193325810254,-3.7766472160421));
#66816=CARTESIAN_POINT('Ctrl Pts',(-23.5090016758881,12.5818064945809,-3.4845162158006));
#66817=CARTESIAN_POINT('Ctrl Pts',(-23.484592830165,12.2004820816042,-3.24720404572943));
#66818=CARTESIAN_POINT('Ctrl Pts',(-23.4464839655589,11.5791039345357,-2.98454272618526));
#66819=CARTESIAN_POINT('Ctrl Pts',(-23.4335068125947,11.3621073396055,-2.91271141912405));
#66820=CARTESIAN_POINT('Ctrl Pts',(-23.3973171935771,10.7367537118015,-2.76006416037631));
#66821=CARTESIAN_POINT('Ctrl Pts',(-23.3746868396262,10.3208579053535,-2.72107458050878));
#66822=CARTESIAN_POINT('Ctrl Pts',(-23.3367605198731,9.64691836463789,-2.75646976697985));
#66823=CARTESIAN_POINT('Ctrl Pts',(-23.3220373816232,9.3897063732441,-2.79367902397596));
#66824=CARTESIAN_POINT('Ctrl Pts',(-23.2925172001717,8.87968350748323,-2.91571422403364));
#66825=CARTESIAN_POINT('Ctrl Pts',(-23.2779320658428,8.62820751784597,-3.00130584031873));
#66826=CARTESIAN_POINT('Ctrl Pts',(-23.2322650016507,7.87791905695821,-3.33750035182252));
#66827=CARTESIAN_POINT('Ctrl Pts',(-23.2006283778644,7.41908692516015,-3.66275820743672));
#66828=CARTESIAN_POINT('Ctrl Pts',(-23.1541830548561,6.84351004176925,-4.26987945763089));
#66829=CARTESIAN_POINT('Ctrl Pts',(-23.138764797502,6.67163085484486,-4.49113043515536));
#66830=CARTESIAN_POINT('Ctrl Pts',(-23.1094026333514,6.39258651629209,-4.93404287435651));
#66831=CARTESIAN_POINT('Ctrl Pts',(-23.0955826074097,6.28049087961493,-5.15126367730691));
#66832=CARTESIAN_POINT('Ctrl Pts',(-23.0502851047814,5.97511370653541,-5.89289766113601));
#66833=CARTESIAN_POINT('Ctrl Pts',(-23.0200794903383,5.8660154708496,-6.44565312269876));
#66834=CARTESIAN_POINT('Ctrl Pts',(-22.9755292798195,5.86670271206618,-7.23455531700981));
#66835=CARTESIAN_POINT('Ctrl Pts',(-22.9624255642123,5.88565354052962,-7.46500360398424));
#66836=CARTESIAN_POINT('Ctrl Pts',(-22.9360178923028,5.96242869756211,-7.93115308143177));
#66837=CARTESIAN_POINT('Ctrl Pts',(-22.9227269527656,6.02187927087701,-8.16575496768535));
#66838=CARTESIAN_POINT('Ctrl Pts',(-22.8885016510635,6.2230623764673,-8.74714389776903));
#66839=CARTESIAN_POINT('Ctrl Pts',(-22.8673967100352,6.39113240840198,-9.08263163558883));
#66840=CARTESIAN_POINT('Ctrl Pts',(-22.8313068463502,6.75008956149188,-9.61220121735023));
#66841=CARTESIAN_POINT('Ctrl Pts',(-22.8166199946301,6.91972932205428,-9.81804642132396));
#66842=CARTESIAN_POINT('Ctrl Pts',(-22.7764052945812,7.43090592911632,-10.3318258316762));
#66843=CARTESIAN_POINT('Ctrl Pts',(-22.7505241782358,7.80470051667608,-10.6026024093102));
#66844=CARTESIAN_POINT('Ctrl Pts',(-22.6994601906312,8.61575317480828,-11.0104340665967));
#66845=CARTESIAN_POINT('Ctrl Pts',(-22.6750348689543,9.0465220160346,-11.1475503300876));
#66846=CARTESIAN_POINT('Ctrl Pts',(-22.6356423579933,9.73858190014085,-11.2524342877029));
#66847=CARTESIAN_POINT('Ctrl Pts',(-22.6214059145636,9.98926909238338,-11.26806137762));
#66848=CARTESIAN_POINT('Ctrl Pts',(-22.5828682290083,10.6746545951026,-11.2503104255814));
#66849=CARTESIAN_POINT('Ctrl Pts',(-22.5592036554187,11.1051607797456,-11.1725799713837));
#66850=CARTESIAN_POINT('Ctrl Pts',(-22.532713960555,11.5504911528519,-11.0193594451106));
#66851=CARTESIAN_POINT('Ctrl Pts',(-22.5306862986621,11.5843873590537,-11.0072144029709));
#66852=CARTESIAN_POINT('Ctrl Pts',(-22.5286570444943,11.618114651272,-10.9946458441291));
#66853=CARTESIAN_POINT('',(-23.533999981871,12.9193850840203,-10.2235360174615));
#66854=CARTESIAN_POINT('Origin',(-23.534,10.1295,-7.));
#66855=CARTESIAN_POINT('',(-22.2043183294109,10.1295365072714,-11.2628938598663));
#66856=CARTESIAN_POINT('Ctrl Pts',(-23.533999981871,12.9193850840203,-10.2235360174615));
#66857=CARTESIAN_POINT('Ctrl Pts',(-23.5009788547478,13.3648360859832,-9.83730561563166));
#66858=CARTESIAN_POINT('Ctrl Pts',(-23.4291758459887,14.1588395586771,-8.79502344007021));
#66859=CARTESIAN_POINT('Ctrl Pts',(-23.3185909555933,14.5604905826756,-6.80076298861617));
#66860=CARTESIAN_POINT('Ctrl Pts',(-23.2022453106852,13.9513208636606,-4.74899583476332));
#66861=CARTESIAN_POINT('Ctrl Pts',(-23.0858996657769,12.452270995998,-3.22136570469558));
#66862=CARTESIAN_POINT('Ctrl Pts',(-22.9695540208687,10.4123750626855,-2.57356516157568));
#66863=CARTESIAN_POINT('Ctrl Pts',(-22.8532083759605,8.30661439543301,-2.9564333045403));
#66864=CARTESIAN_POINT('Ctrl Pts',(-22.7368627310523,6.62530205950465,-4.28082127060911));
#66865=CARTESIAN_POINT('Ctrl Pts',(-22.6205170861441,5.75991783379543,-6.23835174036327));
#66866=CARTESIAN_POINT('Ctrl Pts',(-22.5041714412359,5.9119701463398,-8.37323075593554));
#66867=CARTESIAN_POINT('Ctrl Pts',(-22.3878257963277,7.04603468702391,-10.1883540588533));
#66868=CARTESIAN_POINT('Ctrl Pts',(-22.2878747590527,8.63711446750853,-11.1099400088585));
#66869=CARTESIAN_POINT('Ctrl Pts',(-22.2267056034138,9.72970022779226,-11.2625492465514));
#66870=CARTESIAN_POINT('Ctrl Pts',(-22.2043183294109,10.1295365056039,-11.2626991438894));
#66871=CARTESIAN_POINT('Ctrl Pts',(-22.2043183294109,10.1295365081804,-11.2629999998437));
#66872=CARTESIAN_POINT('Ctrl Pts',(-22.1969189537551,10.2616985400649,-11.2629988680127));
#66873=CARTESIAN_POINT('Ctrl Pts',(-22.1895195780993,10.3938406290833,-11.2568474434062));
#66874=CARTESIAN_POINT('Ctrl Pts',(-22.1821202024435,10.5253950557853,-11.2445772586684));
#66875=CARTESIAN_POINT('Ctrl Pts',(-22.1747186558373,10.6569880800863,-11.2323034739021));
#66876=CARTESIAN_POINT('Ctrl Pts',(-22.1673171092312,10.787992785182,-11.2139073736702));
#66877=CARTESIAN_POINT('Ctrl Pts',(-22.159915562625,10.9178466698904,-11.1894723448273));
#66878=CARTESIAN_POINT('Ctrl Pts',(-22.1583218772538,10.9458065338847,-11.1842110460631));
#66879=CARTESIAN_POINT('Ctrl Pts',(-22.1567281918825,10.9737130747606,-11.1786699613312));
#66880=CARTESIAN_POINT('Ctrl Pts',(-22.1551345065113,11.0015607336212,-11.1728502341776));
#66881=CARTESIAN_POINT('Ctrl Pts',(-22.1478857890208,11.1282230068014,-11.1463797910337));
#66882=CARTESIAN_POINT('Ctrl Pts',(-22.1406370715302,11.2537022086528,-11.1141332404387));
#66883=CARTESIAN_POINT('Ctrl Pts',(-22.1333883540397,11.3774686349185,-11.0762413184525));
#66884=CARTESIAN_POINT('Ctrl Pts',(-22.1286445389192,11.4584657278658,-11.0514435148828));
#66885=CARTESIAN_POINT('Ctrl Pts',(-22.1239007237987,11.5387294697866,-11.0242289282653));
#66886=CARTESIAN_POINT('Ctrl Pts',(-22.1191569086782,11.6181146495903,-10.9946458447559));
#66887=CARTESIAN_POINT('Origin',(-18.734,-18.952,0.));
#66888=CARTESIAN_POINT('',(-20.7225805821494,-19.6781103692267,-21.2464098430158));
#66889=CARTESIAN_POINT('',(-20.722580582091,-19.6781103693865,-21.465822579505));
#66890=CARTESIAN_POINT('',(-20.7225805821191,-19.6781103693095,0.));
#66891=CARTESIAN_POINT('',(-20.8509993841958,-18.953614718169,-21.5109437210328));
#66892=CARTESIAN_POINT('Ctrl Pts',(-20.722580582091,-19.6781103693865,-21.465822579505));
#66893=CARTESIAN_POINT('Ctrl Pts',(-20.7235155796043,-19.6755497147289,
-21.4659707954636));
#66894=CARTESIAN_POINT('Ctrl Pts',(-20.7244456404574,-19.6729872286501,
-21.4661190479908));
#66895=CARTESIAN_POINT('Ctrl Pts',(-20.7392637896057,-19.6319133320967,
-21.4684943566896));
#66896=CARTESIAN_POINT('Ctrl Pts',(-20.752036519493,-19.5930097144133,-21.4707296572491));
#66897=CARTESIAN_POINT('Ctrl Pts',(-20.7690503572088,-19.5356239558152,
-21.4740356753045));
#66898=CARTESIAN_POINT('Ctrl Pts',(-20.7741842861848,-19.5174157143311,
-21.4750859568108));
#66899=CARTESIAN_POINT('Ctrl Pts',(-20.7947015602454,-19.4407274461673,
-21.4795238028831));
#66900=CARTESIAN_POINT('Ctrl Pts',(-20.8078182966199,-19.3816762398259,
-21.4829755341861));
#66901=CARTESIAN_POINT('Ctrl Pts',(-20.8199726159277,-19.3132330043184,
-21.4870989280524));
#66902=CARTESIAN_POINT('Ctrl Pts',(-20.8214990062904,-19.3043051658438,
-21.4876391708838));
#66903=CARTESIAN_POINT('Ctrl Pts',(-20.8236943731102,-19.2909490836379,
-21.4884513018792));
#66904=CARTESIAN_POINT('Ctrl Pts',(-20.8244066869518,-19.2865279309743,
-21.4887207763421));
#66905=CARTESIAN_POINT('Ctrl Pts',(-20.8256596197291,-19.2785910105057,
-21.4892057453182));
#66906=CARTESIAN_POINT('Ctrl Pts',(-20.8262054097228,-19.2750761148281,
-21.4894209425139));
#66907=CARTESIAN_POINT('Ctrl Pts',(-20.8272520454122,-19.2682218781208,
-21.4898414207746));
#66908=CARTESIAN_POINT('Ctrl Pts',(-20.8277537589423,-19.2648827230304,
-21.4900466455382));
#66909=CARTESIAN_POINT('Ctrl Pts',(-20.8288495023066,-19.257469335688,-21.4905030984026));
#66910=CARTESIAN_POINT('Ctrl Pts',(-20.8294396375628,-19.2533945537653,
-21.4907545413552));
#66911=CARTESIAN_POINT('Ctrl Pts',(-20.8308795084341,-19.2432438265539,
-21.4913822453917));
#66912=CARTESIAN_POINT('Ctrl Pts',(-20.8317147195046,-19.2371659041556,
-21.4917592813314));
#66913=CARTESIAN_POINT('Ctrl Pts',(-20.835602193926,-19.2079347725518,-21.4935780223869));
#66914=CARTESIAN_POINT('Ctrl Pts',(-20.8382974849493,-19.1847367233153,
-21.4950377275373));
#66915=CARTESIAN_POINT('Ctrl Pts',(-20.8474812907066,-19.0923897727793,
-21.5009009877621));
#66916=CARTESIAN_POINT('Ctrl Pts',(-20.8509485267258,-19.0229896553394,
-21.5054226551349));
#66917=CARTESIAN_POINT('Ctrl Pts',(-20.8509994311328,-18.953551961105,-21.509989519712));
#66918=CARTESIAN_POINT('',(-17.1140743056113,-20.3149122292574,-22.));
#66919=CARTESIAN_POINT('Ctrl Pts',(-20.8509993841958,-18.953614718169,-21.5109437210328));
#66920=CARTESIAN_POINT('Ctrl Pts',(-20.8510560133107,-18.8793703058911,
-21.5154240901546));
#66921=CARTESIAN_POINT('Ctrl Pts',(-20.8472020782088,-18.804981409641,-21.5199044592764));
#66922=CARTESIAN_POINT('Ctrl Pts',(-20.8394225349145,-18.7309005891588,
-21.5243848283982));
#66923=CARTESIAN_POINT('Ctrl Pts',(-20.8319236702397,-18.6594925351418,
-21.5287035500076));
#66924=CARTESIAN_POINT('Ctrl Pts',(-20.820777658289,-18.5883712544674,-21.5330222716171));
#66925=CARTESIAN_POINT('Ctrl Pts',(-20.8060239432422,-18.5179426551354,
-21.5373409932266));
#66926=CARTESIAN_POINT('Ctrl Pts',(-20.791280056931,-18.4475609744317,-21.5416568377592));
#66927=CARTESIAN_POINT('Ctrl Pts',(-20.7729333337529,-18.3778715449745,
-21.5459726822918));
#66928=CARTESIAN_POINT('Ctrl Pts',(-20.7510747171251,-18.3092725417919,
-21.5502885268244));
#66929=CARTESIAN_POINT('Ctrl Pts',(-20.7292229915306,-18.2406951647726,
-21.5546030107664));
#66930=CARTESIAN_POINT('Ctrl Pts',(-20.7038617199401,-18.1732080048576,
-21.5589174947085));
#66931=CARTESIAN_POINT('Ctrl Pts',(-20.6751318662711,-18.1071946509717,
-21.5632319786505));
#66932=CARTESIAN_POINT('Ctrl Pts',(-20.646400988223,-18.0411789433423,-21.5675466164279));
#66933=CARTESIAN_POINT('Ctrl Pts',(-20.6143014909514,-17.9766376000802,
-21.5718612542053));
#66934=CARTESIAN_POINT('Ctrl Pts',(-20.5790219474228,-17.9139330399593,
-21.5761758919827));
#66935=CARTESIAN_POINT('Ctrl Pts',(-20.5437075154313,-17.8511664703707,
-21.5804947965692));
#66936=CARTESIAN_POINT('Ctrl Pts',(-20.5052070087195,-17.7902407402828,
-21.5848137011558));
#66937=CARTESIAN_POINT('Ctrl Pts',(-20.4637537458688,-17.7314915081602,
-21.5891326057424));
#66938=CARTESIAN_POINT('Ctrl Pts',(-20.4222758278492,-17.6727073337405,
-21.593454079085));
#66939=CARTESIAN_POINT('Ctrl Pts',(-20.3778419690816,-17.6161026206995,
-21.5977755524276));
#66940=CARTESIAN_POINT('Ctrl Pts',(-20.3307256571012,-17.561979792969,-21.6020970257703));
#66941=CARTESIAN_POINT('Ctrl Pts',(-20.2835347568318,-17.507771285164,-21.6064253402958));
#66942=CARTESIAN_POINT('Ctrl Pts',(-20.2336532809969,-17.4560528519306,
-21.6107536548212));
#66943=CARTESIAN_POINT('Ctrl Pts',(-20.1813905809776,-17.4070891591754,
-21.6150819693466));
#66944=CARTESIAN_POINT('Ctrl Pts',(-20.1677438166228,-17.3943038270605,
-21.616212172883));
#66945=CARTESIAN_POINT('Ctrl Pts',(-20.1539348588654,-17.3817060999665,
-21.6173423764194));
#66946=CARTESIAN_POINT('Ctrl Pts',(-20.1399695509607,-17.369300211104,-21.6184725799558));
#66947=CARTESIAN_POINT('Ctrl Pts',(-20.0856805133166,-17.3210732925096,
-21.6228661574372));
#66948=CARTESIAN_POINT('Ctrl Pts',(-20.0288041823845,-17.2755513561322,
-21.6272597349186));
#66949=CARTESIAN_POINT('Ctrl Pts',(-19.969640873017,-17.2330233762701,-21.6316533124001));
#66950=CARTESIAN_POINT('Ctrl Pts',(-19.9105638618643,-17.1905574295968,
-21.6360404812154));
#66951=CARTESIAN_POINT('Ctrl Pts',(-19.849206882515,-17.1510770477242,-21.6404276500308));
#66952=CARTESIAN_POINT('Ctrl Pts',(-19.7859046048043,-17.1148321518186,
-21.6448148188462));
#66953=CARTESIAN_POINT('Ctrl Pts',(-19.7226747936877,-17.0786287480086,
-21.6491969653592));
#66954=CARTESIAN_POINT('Ctrl Pts',(-19.6575045236034,-17.0456537097674,
-21.6535791118721));
#66955=CARTESIAN_POINT('Ctrl Pts',(-19.5907574447862,-17.0161137221408,
-21.6579612583851));
#66956=CARTESIAN_POINT('Ctrl Pts',(-19.524051506928,-16.9865919421039,-21.6623407038703));
#66957=CARTESIAN_POINT('Ctrl Pts',(-19.4557711276412,-16.960501205489,-21.6667201493556));
#66958=CARTESIAN_POINT('Ctrl Pts',(-19.3863033026644,-16.9380016382,-21.6710995948408));
#66959=CARTESIAN_POINT('Ctrl Pts',(-19.3168555527303,-16.9155085729106,
-21.6754777747394));
#66960=CARTESIAN_POINT('Ctrl Pts',(-19.2462214956912,-16.8966047644762,
-21.6798559546379));
#66961=CARTESIAN_POINT('Ctrl Pts',(-19.1748052243022,-16.8814011121833,
-21.6842341345365));
#66962=CARTESIAN_POINT('Ctrl Pts',(-19.10338621101,-16.8661968761726,-21.6886124825276));
#66963=CARTESIAN_POINT('Ctrl Pts',(-19.0311853945028,-16.8546931765608,
-21.6929908305188));
#66964=CARTESIAN_POINT('Ctrl Pts',(-18.958617414822,-16.8469498778037,-21.6973691785099));
#66965=CARTESIAN_POINT('Ctrl Pts',(-18.8859734847581,-16.8391984748317,
-21.7017521089244));
#66966=CARTESIAN_POINT('Ctrl Pts',(-18.8129621034892,-16.835215381558,-21.7061350393389));
#66967=CARTESIAN_POINT('Ctrl Pts',(-18.7400025813939,-16.8350085099329,
-21.7105179697534));
#66968=CARTESIAN_POINT('Ctrl Pts',(-18.6670027054265,-16.8348015238872,
-21.7149033243644));
#66969=CARTESIAN_POINT('Ctrl Pts',(-18.5940552263849,-16.8383748946447,
-21.7192886789753));
#66970=CARTESIAN_POINT('Ctrl Pts',(-18.5215762918332,-16.8456844566379,
-21.7236740335863));
#66971=CARTESIAN_POINT('Ctrl Pts',(-18.4489692699444,-16.8530069363477,
-21.728067138151));
#66972=CARTESIAN_POINT('Ctrl Pts',(-18.3768329218414,-16.8640787198162,
-21.7324602427158));
#66973=CARTESIAN_POINT('Ctrl Pts',(-18.3055745682925,-16.8788042423673,
-21.7368533472805));
#66974=CARTESIAN_POINT('Ctrl Pts',(-18.2580212556926,-16.8886311235987,
-21.739785027066));
#66975=CARTESIAN_POINT('Ctrl Pts',(-18.2108587080193,-16.900084095337,-21.7427167068516));
#66976=CARTESIAN_POINT('Ctrl Pts',(-18.1642037039559,-16.913122568418,-21.7456483866372));
#66977=CARTESIAN_POINT('Ctrl Pts',(-18.0951065059757,-16.932432864793,-21.7499902758433));
#66978=CARTESIAN_POINT('Ctrl Pts',(-18.0268409185985,-16.9553020920462,
-21.7543321650495));
#66979=CARTESIAN_POINT('Ctrl Pts',(-17.9598056269363,-16.9816416385042,
-21.7586740542557));
#66980=CARTESIAN_POINT('Ctrl Pts',(-17.8928712802768,-17.007941521592,-21.7630094052339));
#66981=CARTESIAN_POINT('Ctrl Pts',(-17.8271640088704,-17.0377011783514,
-21.7673447562122));
#66982=CARTESIAN_POINT('Ctrl Pts',(-17.7630690182321,-17.0707817700641,
-21.7716801071904));
#66983=CARTESIAN_POINT('Ctrl Pts',(-17.6990476945068,-17.1038243409416,
-21.7760104753779));
#66984=CARTESIAN_POINT('Ctrl Pts',(-17.6366354094004,-17.140180045608,-21.7803408435655));
#66985=CARTESIAN_POINT('Ctrl Pts',(-17.576197298269,-17.1796620232404,-21.784671211753));
#66986=CARTESIAN_POINT('Ctrl Pts',(-17.5157963311547,-17.2191197360633,
-21.7889989185855));
#66987=CARTESIAN_POINT('Ctrl Pts',(-17.4573675446825,-17.2616996436244,
-21.793326625418));
#66988=CARTESIAN_POINT('Ctrl Pts',(-17.4012499559382,-17.3071698202996,
-21.7976543322506));
#66989=CARTESIAN_POINT('Ctrl Pts',(-17.3451474140536,-17.3526278050152,
-21.8019808786911));
#66990=CARTESIAN_POINT('Ctrl Pts',(-17.2913552237362,-17.4009742110386,
-21.8063074251317));
#66991=CARTESIAN_POINT('Ctrl Pts',(-17.2401804886106,-17.4519359122383,
-21.8106339715723));
#66992=CARTESIAN_POINT('Ctrl Pts',(-17.1890017454992,-17.502901604739,-21.8149608568663));
#66993=CARTESIAN_POINT('Ctrl Pts',(-17.1404412125279,-17.5564826492106,
-21.8192877421603));
#66994=CARTESIAN_POINT('Ctrl Pts',(-17.0947688687351,-17.6123693425829,
-21.8236146274544));
#66995=CARTESIAN_POINT('Ctrl Pts',(-17.0490417134499,-17.6683231057134,
-21.8279467054541));
#66996=CARTESIAN_POINT('Ctrl Pts',(-17.0062099790967,-17.7265876580954,
-21.8322787834538));
#66997=CARTESIAN_POINT('Ctrl Pts',(-16.9665025074284,-17.7868212095334,
-21.8366108614535));
#66998=CARTESIAN_POINT('Ctrl Pts',(-16.9267705288898,-17.8470919362378,
-21.8409456131484));
#66999=CARTESIAN_POINT('Ctrl Pts',(-16.8901668972173,-17.9093336530359,
-21.8452803648433));
#67000=CARTESIAN_POINT('Ctrl Pts',(-16.8568748225048,-17.9731792462286,
-21.8496151165381));
#67001=CARTESIAN_POINT('Ctrl Pts',(-16.8235156981184,-18.0371534233633,
-21.8539585983494));
#67002=CARTESIAN_POINT('Ctrl Pts',(-16.7934816509746,-18.1027374769631,
-21.8583020801606));
#67003=CARTESIAN_POINT('Ctrl Pts',(-16.7669077870852,-18.1695441061056,
-21.8626455619719));
#67004=CARTESIAN_POINT('Ctrl Pts',(-16.7461498194961,-18.221729586104,-21.8660384390875));
#67005=CARTESIAN_POINT('Ctrl Pts',(-16.7275022238381,-18.2746606281223,
-21.869431316203));
#67006=CARTESIAN_POINT('Ctrl Pts',(-16.7110077838934,-18.328147859207,-21.8728241933186));
#67007=CARTESIAN_POINT('Ctrl Pts',(-16.6890805388882,-18.3992522813377,
-21.8773345888236));
#67008=CARTESIAN_POINT('Ctrl Pts',(-16.6708712302021,-18.471627433023,-21.8818449843287));
#67009=CARTESIAN_POINT('Ctrl Pts',(-16.65651913225,-18.5448609032129,-21.8863553798337));
#67010=CARTESIAN_POINT('Ctrl Pts',(-16.6414517292682,-18.6217443115328,
-21.8910905723407));
#67011=CARTESIAN_POINT('Ctrl Pts',(-16.6306362647773,-18.699573380232,-21.8958257648476));
#67012=CARTESIAN_POINT('Ctrl Pts',(-16.6241750600365,-18.7778514349529,
-21.9005609573545));
#67013=CARTESIAN_POINT('Ctrl Pts',(-16.6180410539461,-18.8521654497015,
-21.9050563573367));
#67014=CARTESIAN_POINT('Ctrl Pts',(-16.6158311159158,-18.9268835670766,
-21.9095517573189));
#67015=CARTESIAN_POINT('Ctrl Pts',(-16.6175804464527,-19.001570892293,-21.9140471573011));
#67016=CARTESIAN_POINT('Ctrl Pts',(-16.6193281321099,-19.0761879896894,
-21.9185383302991));
#67017=CARTESIAN_POINT('Ctrl Pts',(-16.6250276759246,-19.1507739043837,
-21.9230295032971));
#67018=CARTESIAN_POINT('Ctrl Pts',(-16.6346622676094,-19.2248920763987,
-21.9275206762951));
#67019=CARTESIAN_POINT('Ctrl Pts',(-16.6442903170874,-19.2989599197204,
-21.932008799638));
#67020=CARTESIAN_POINT('Ctrl Pts',(-16.6578480436051,-19.3725602066461,
-21.9364969229808));
#67021=CARTESIAN_POINT('Ctrl Pts',(-16.6752667781491,-19.4452611085899,
-21.9409850463236));
#67022=CARTESIAN_POINT('Ctrl Pts',(-16.6926782312815,-19.5179316199686,
-21.9454712935328));
#67023=CARTESIAN_POINT('Ctrl Pts',(-16.7139473766674,-19.5897030572418,
-21.949957540742));
#67024=CARTESIAN_POINT('Ctrl Pts',(-16.7389546395216,-19.6601546509298,
-21.9544437879513));
#67025=CARTESIAN_POINT('Ctrl Pts',(-16.7639650091895,-19.7306149972742,
-21.9589305925159));
#67026=CARTESIAN_POINT('Ctrl Pts',(-16.792714280612,-19.7997547457854,-21.9634173970806));
#67027=CARTESIAN_POINT('Ctrl Pts',(-16.8250335623977,-19.8671700061235,
-21.9679042016453));
#67028=CARTESIAN_POINT('Ctrl Pts',(-16.8573543979593,-19.9345885075052,
-21.9723912219168));
#67029=CARTESIAN_POINT('Ctrl Pts',(-16.8932453841005,-20.0002819530908,
-21.9768782421882));
#67030=CARTESIAN_POINT('Ctrl Pts',(-16.9324909433493,-20.0638696500964,
-21.9813652624597));
#67031=CARTESIAN_POINT('Ctrl Pts',(-16.971763585854,-20.1275012288023,-21.9858553792119));
#67032=CARTESIAN_POINT('Ctrl Pts',(-17.0143951804746,-20.1890237784353,
-21.9903454959641));
#67033=CARTESIAN_POINT('Ctrl Pts',(-17.0601263939598,-20.2480849320172,
-21.9948356127163));
#67034=CARTESIAN_POINT('Ctrl Pts',(-17.0776592489258,-20.2707283425231,
-21.9965570751442));
#67035=CARTESIAN_POINT('Ctrl Pts',(-17.0956472766607,-20.2930102923405,
-21.9982785375721));
#67036=CARTESIAN_POINT('Ctrl Pts',(-17.1140743056112,-20.3149122292573,
-22.));
#67037=CARTESIAN_POINT('',(-20.3539401105369,-20.3148950943758,-21.9999997808643));
#67038=CARTESIAN_POINT('Origin',(-18.734,-18.952,-22.));
#67039=CARTESIAN_POINT('',(-20.8509997094769,-18.9531090873175,-21.2890562790225));
#67040=CARTESIAN_POINT('Ctrl Pts',(-20.3539401105369,-20.3148950943758,
-21.9999997808643));
#67041=CARTESIAN_POINT('Ctrl Pts',(-20.3072932296543,-20.3703396797185,
-21.9956147616661));
#67042=CARTESIAN_POINT('Ctrl Pts',(-20.2577049138449,-20.4234955896159,
-21.9912297424679));
#67043=CARTESIAN_POINT('Ctrl Pts',(-20.2054285432655,-20.4740338504986,
-21.9868447232696));
#67044=CARTESIAN_POINT('Ctrl Pts',(-20.1532297926735,-20.5244970721403,
-21.9824662149506));
#67045=CARTESIAN_POINT('Ctrl Pts',(-20.0983512546661,-20.5723500270703,
-21.9780877066316));
#67046=CARTESIAN_POINT('Ctrl Pts',(-20.0410860694924,-20.6172972728431,
-21.9737091983125));
#67047=CARTESIAN_POINT('Ctrl Pts',(-19.983888278367,-20.6621916212607,-21.9693358429569));
#67048=CARTESIAN_POINT('Ctrl Pts',(-19.9243097978752,-20.7041867567888,
-21.9649624876012));
#67049=CARTESIAN_POINT('Ctrl Pts',(-19.8626788010172,-20.7430257296126,
-21.9605891322455));
#67050=CARTESIAN_POINT('Ctrl Pts',(-19.8010868010387,-20.7818401271607,
-21.956218544121));
#67051=CARTESIAN_POINT('Ctrl Pts',(-19.7374452692593,-20.8175020674031,
-21.9518479559964));
#67052=CARTESIAN_POINT('Ctrl Pts',(-19.6721123140465,-20.8497972194717,
-21.9474773678718));
#67053=CARTESIAN_POINT('Ctrl Pts',(-19.6067990615792,-20.8820826321498,
-21.9431080978047));
#67054=CARTESIAN_POINT('Ctrl Pts',(-19.5397958312689,-20.911003058507,-21.9387388277375));
#67055=CARTESIAN_POINT('Ctrl Pts',(-19.4714848515874,-20.9363903581904,
-21.9343695576704));
#67056=CARTESIAN_POINT('Ctrl Pts',(-19.4031718505269,-20.9617784091052,
-21.9300001583129));
#67057=CARTESIAN_POINT('Ctrl Pts',(-19.3335514769124,-20.9836329595348,
-21.9256307589554));
#67058=CARTESIAN_POINT('Ctrl Pts',(-19.2630238363122,-21.001834817885,-21.9212613595979));
#67059=CARTESIAN_POINT('Ctrl Pts',(-19.192424400798,-21.0200552051529,-21.9168875123296));
#67060=CARTESIAN_POINT('Ctrl Pts',(-19.1209163233831,-21.0346153567022,
-21.9125136650614));
#67061=CARTESIAN_POINT('Ctrl Pts',(-19.0489118445282,-21.0454468061491,
-21.9081398177931));
#67062=CARTESIAN_POINT('Ctrl Pts',(-18.9768675429743,-21.0562842460226,
-21.9037635515308));
#67063=CARTESIAN_POINT('Ctrl Pts',(-18.904326774497,-21.0633888314031,-21.8993872852686));
#67064=CARTESIAN_POINT('Ctrl Pts',(-18.8317061863209,-21.0667440746234,
-21.8950110190063));
#67065=CARTESIAN_POINT('Ctrl Pts',(-18.7589614597164,-21.0701050533332,
-21.8906272719066));
#67066=CARTESIAN_POINT('Ctrl Pts',(-18.6861371242322,-21.0697038968461,
-21.8862435248068));
#67067=CARTESIAN_POINT('Ctrl Pts',(-18.6136484217024,-21.0655762341589,
-21.8818597777071));
#67068=CARTESIAN_POINT('Ctrl Pts',(-18.5716418570464,-21.063184289987,-21.8793194348736));
#67069=CARTESIAN_POINT('Ctrl Pts',(-18.5297478967642,-21.0595419177169,
-21.8767790920401));
#67070=CARTESIAN_POINT('Ctrl Pts',(-18.4880458377735,-21.0546639175302,
-21.8742387492067));
#67071=CARTESIAN_POINT('Ctrl Pts',(-18.4158851680032,-21.0462230930451,
-21.8698429748793));
#67072=CARTESIAN_POINT('Ctrl Pts',(-18.3440241776343,-21.0340474650401,
-21.8654472005519));
#67073=CARTESIAN_POINT('Ctrl Pts',(-18.2728787135213,-21.0181694410566,
-21.8610514262245));
#67074=CARTESIAN_POINT('Ctrl Pts',(-18.2018360755882,-21.0023143655011,
-21.8566620050875));
#67075=CARTESIAN_POINT('Ctrl Pts',(-18.1315073759669,-20.9827676217893,
-21.8522725839506));
#67076=CARTESIAN_POINT('Ctrl Pts',(-18.0623020985936,-20.9596132419483,
-21.8478831628136));
#67077=CARTESIAN_POINT('Ctrl Pts',(-17.9931748381961,-20.9364849646642,
-21.8434986899895));
#67078=CARTESIAN_POINT('Ctrl Pts',(-17.9251689375377,-20.9097572825852,
-21.8391142171653));
#67079=CARTESIAN_POINT('Ctrl Pts',(-17.8586808325707,-20.8795646176279,
-21.8347297443412));
#67080=CARTESIAN_POINT('Ctrl Pts',(-17.7922330111159,-20.8493902456658,
-21.8303479279616));
#67081=CARTESIAN_POINT('Ctrl Pts',(-17.7273015969599,-20.8157552549639,
-21.8259661115821));
#67082=CARTESIAN_POINT('Ctrl Pts',(-17.6642637491768,-20.7788424545304,
-21.8215842952025));
#67083=CARTESIAN_POINT('Ctrl Pts',(-17.6012435076605,-20.7419399637226,
-21.8172037026501));
#67084=CARTESIAN_POINT('Ctrl Pts',(-17.5401161967491,-20.7017617236165,
-21.8128231100976));
#67085=CARTESIAN_POINT('Ctrl Pts',(-17.4812335587017,-20.6585360364073,
-21.8084425175452));
#67086=CARTESIAN_POINT('Ctrl Pts',(-17.4223481372602,-20.6153083059113,
-21.8040617179213));
#67087=CARTESIAN_POINT('Ctrl Pts',(-17.3657079854645,-20.5690331281733,
-21.7996809182973));
#67088=CARTESIAN_POINT('Ctrl Pts',(-17.3116337298584,-20.5199806100726,
-21.7953001186734));
#67089=CARTESIAN_POINT('Ctrl Pts',(-17.2575023549029,-20.47087627715,-21.790914691553));
#67090=CARTESIAN_POINT('Ctrl Pts',(-17.2059426440142,-20.4189890701121,
-21.7865292644327));
#67091=CARTESIAN_POINT('Ctrl Pts',(-17.1572395226006,-20.3646271259293,
-21.7821438373123));
#67092=CARTESIAN_POINT('Ctrl Pts',(-17.1085091560373,-20.3102347709788,
-21.7777559569279));
#67093=CARTESIAN_POINT('Ctrl Pts',(-17.0626388625667,-20.253365296582,-21.7733680765434));
#67094=CARTESIAN_POINT('Ctrl Pts',(-17.0198725666879,-20.1943591036278,
-21.768980196159));
#67095=CARTESIAN_POINT('Ctrl Pts',(-16.9770305343292,-20.1352484143348,
-21.7645845451083));
#67096=CARTESIAN_POINT('Ctrl Pts',(-16.9373037385248,-20.0739938533524,
-21.7601888940575));
#67097=CARTESIAN_POINT('Ctrl Pts',(-16.9008918467625,-20.010963407552,-21.7557932430068));
#67098=CARTESIAN_POINT('Ctrl Pts',(-16.8767856902822,-19.9692346833373,
-21.7528831428463));
#67099=CARTESIAN_POINT('Ctrl Pts',(-16.8541315013796,-19.9267281135982,
-21.7499730426858));
#67100=CARTESIAN_POINT('Ctrl Pts',(-16.8329755935997,-19.8835552620593,
-21.7470629425253));
#67101=CARTESIAN_POINT('Ctrl Pts',(-16.8011149796973,-19.8185373215268,
-21.7426803568856));
#67102=CARTESIAN_POINT('Ctrl Pts',(-16.7725300723094,-19.7517529070192,
-21.7382977712459));
#67103=CARTESIAN_POINT('Ctrl Pts',(-16.7474199334088,-19.6835658815327,
-21.7339151856062));
#67104=CARTESIAN_POINT('Ctrl Pts',(-16.722347574114,-19.6154814472323,-21.7295391938112));
#67105=CARTESIAN_POINT('Ctrl Pts',(-16.7007397717712,-19.5459990409051,
-21.7251632020162));
#67106=CARTESIAN_POINT('Ctrl Pts',(-16.6827489097976,-19.4755054583704,
-21.7207872102213));
#67107=CARTESIAN_POINT('Ctrl Pts',(-16.6647796017072,-19.4050963304016,
-21.7164164610665));
#67108=CARTESIAN_POINT('Ctrl Pts',(-16.6504187455061,-19.3336788989525,
-21.7120457119117));
#67109=CARTESIAN_POINT('Ctrl Pts',(-16.6397693978102,-19.2616565595166,
-21.7076749627569));
#67110=CARTESIAN_POINT('Ctrl Pts',(-16.6291269464843,-19.1896808607495,
-21.7033070440387));
#67111=CARTESIAN_POINT('Ctrl Pts',(-16.6221913058276,-19.117101508527,-21.6989391253204));
#67112=CARTESIAN_POINT('Ctrl Pts',(-16.6190144751312,-19.0443321698839,
-21.6945712066022));
#67113=CARTESIAN_POINT('Ctrl Pts',(-16.6158386463066,-18.9715857803861,
-21.6902046653873));
#67114=CARTESIAN_POINT('Ctrl Pts',(-16.6164192953802,-18.8986500064394,
-21.6858381241723));
#67115=CARTESIAN_POINT('Ctrl Pts',(-16.6207564302585,-18.8259420175236,
-21.6814715829573));
#67116=CARTESIAN_POINT('Ctrl Pts',(-16.6250936381862,-18.7532328040023,
-21.6771049681976));
#67117=CARTESIAN_POINT('Ctrl Pts',(-16.6331874267156,-18.6807518659564,
-21.6727383534379));
#67118=CARTESIAN_POINT('Ctrl Pts',(-16.64498579739,-18.6089130412075,-21.6683717386782));
#67119=CARTESIAN_POINT('Ctrl Pts',(-16.6567963801275,-18.5369998587107,
-21.6640006041948));
#67120=CARTESIAN_POINT('Ctrl Pts',(-16.672319122297,-18.465730594939,-21.6596294697114));
#67121=CARTESIAN_POINT('Ctrl Pts',(-16.6914506939752,-18.3955098091991,
-21.655258335228));
#67122=CARTESIAN_POINT('Ctrl Pts',(-16.7105926424343,-18.325250936379,-21.6508848298832));
#67123=CARTESIAN_POINT('Ctrl Pts',(-16.7333471660201,-18.2560421336627,
-21.6465113245384));
#67124=CARTESIAN_POINT('Ctrl Pts',(-16.7595615727462,-18.1882710579117,
-21.6421378191936));
#67125=CARTESIAN_POINT('Ctrl Pts',(-16.7858227154186,-18.1203791575545,
-21.6377565166129));
#67126=CARTESIAN_POINT('Ctrl Pts',(-16.8155558613104,-18.0539305447508,
-21.6333752140323));
#67127=CARTESIAN_POINT('Ctrl Pts',(-16.8485611226492,-17.9892906774244,
-21.6289939114516));
#67128=CARTESIAN_POINT('Ctrl Pts',(-16.8714288660015,-17.9445048512745,
-21.6259583195824));
#67129=CARTESIAN_POINT('Ctrl Pts',(-16.8958663903147,-17.9005867928719,
-21.6229227277131));
#67130=CARTESIAN_POINT('Ctrl Pts',(-16.9217951734766,-17.8576496599694,
-21.6198871358438));
#67131=CARTESIAN_POINT('Ctrl Pts',(-16.9592871125939,-17.7955643564438,
-21.6154977965973));
#67132=CARTESIAN_POINT('Ctrl Pts',(-17.0000461986468,-17.7352871847913,
-21.6111084573508));
#67133=CARTESIAN_POINT('Ctrl Pts',(-17.0438726443021,-17.6771829458619,
-21.6067191181042));
#67134=CARTESIAN_POINT('Ctrl Pts',(-17.0876341035589,-17.6191648646202,
-21.6023362874245));
#67135=CARTESIAN_POINT('Ctrl Pts',(-17.134453605312,-17.5633137014982,-21.5979534567447));
#67136=CARTESIAN_POINT('Ctrl Pts',(-17.1840868960386,-17.5099672783988,
-21.593570626065));
#67137=CARTESIAN_POINT('Ctrl Pts',(-17.2336618872153,-17.4566835163159,
-21.5891929434835));
#67138=CARTESIAN_POINT('Ctrl Pts',(-17.2860437748972,-17.4058990008948,
-21.5848152609019));
#67139=CARTESIAN_POINT('Ctrl Pts',(-17.3409477315906,-17.3579189551721,
-21.5804375783204));
#67140=CARTESIAN_POINT('Ctrl Pts',(-17.3958168761313,-17.3099693314588,
-21.5760626714324));
#67141=CARTESIAN_POINT('Ctrl Pts',(-17.4532045546155,-17.2648209656694,
-21.5716877645444));
#67142=CARTESIAN_POINT('Ctrl Pts',(-17.5127897524411,-17.2227416239159,
-21.5673128576563));
#67143=CARTESIAN_POINT('Ctrl Pts',(-17.5723567979443,-17.1806751014162,
-21.5629392835611));
#67144=CARTESIAN_POINT('Ctrl Pts',(-17.6341196401156,-17.14167602466,-21.5585657094658));
#67145=CARTESIAN_POINT('Ctrl Pts',(-17.6977262557446,-17.1059702800424,
-21.5541921353705));
#67146=CARTESIAN_POINT('Ctrl Pts',(-17.761334446059,-17.0702636514709,-21.5498184530003));
#67147=CARTESIAN_POINT('Ctrl Pts',(-17.8267860790938,-17.0378507511553,
-21.5454447706301));
#67148=CARTESIAN_POINT('Ctrl Pts',(-17.8937038483149,-17.0089118966287,
-21.5410710882598));
#67149=CARTESIAN_POINT('Ctrl Pts',(-17.9606908447099,-16.9799431045363,
-21.5366928812667));
#67150=CARTESIAN_POINT('Ctrl Pts',(-18.0291465621343,-16.9544557255711,
-21.5323146742736));
#67151=CARTESIAN_POINT('Ctrl Pts',(-18.0986737635119,-16.9325818726103,
-21.5279364672805));
#67152=CARTESIAN_POINT('Ctrl Pts',(-18.168238835056,-16.9106961053709,-21.5235558755599));
#67153=CARTESIAN_POINT('Ctrl Pts',(-18.2388760855,-16.8924279037581,-21.5191752838393));
#67154=CARTESIAN_POINT('Ctrl Pts',(-18.3101757995837,-16.8778587205445,
-21.5147946921187));
#67155=CARTESIAN_POINT('Ctrl Pts',(-18.38160150593,-16.8632637924259,-21.5104063595443));
#67156=CARTESIAN_POINT('Ctrl Pts',(-18.453691536507,-16.8523810078683,-21.5060180269699));
#67157=CARTESIAN_POINT('Ctrl Pts',(-18.5260293173379,-16.8452401192464,
-21.5016296943955));
#67158=CARTESIAN_POINT('Ctrl Pts',(-18.5750331047421,-16.8404026666194,
-21.4986569059845));
#67159=CARTESIAN_POINT('Ctrl Pts',(-18.6241504958208,-16.8372813242577,
-21.4956841175734));
#67160=CARTESIAN_POINT('Ctrl Pts',(-18.6732524736177,-16.8358717576578,
-21.4927113291624));
#67161=CARTESIAN_POINT('Ctrl Pts',(-18.7457477453063,-16.833790641617,-21.4883222370484));
#67162=CARTESIAN_POINT('Ctrl Pts',(-18.8184909189991,-16.8354351540471,
-21.4839331449344));
#67163=CARTESIAN_POINT('Ctrl Pts',(-18.8910671368434,-16.8408347022263,
-21.4795440528204));
#67164=CARTESIAN_POINT('Ctrl Pts',(-18.9635359887558,-16.8462262625614,
-21.4751614537282));
#67165=CARTESIAN_POINT('Ctrl Pts',(-19.0358378982521,-16.8553617955042,
-21.470778854636));
#67166=CARTESIAN_POINT('Ctrl Pts',(-19.1075566334651,-16.8682187155092,
-21.4663962555438));
#67167=CARTESIAN_POINT('Ctrl Pts',(-19.1791915242117,-16.8810606048308,
-21.4620187800316));
#67168=CARTESIAN_POINT('Ctrl Pts',(-19.2502441227826,-16.8976151540491,
-21.4576413045195));
#67169=CARTESIAN_POINT('Ctrl Pts',(-19.3203036537857,-16.9178080165438,
-21.4532638290073));
#67170=CARTESIAN_POINT('Ctrl Pts',(-19.3903190046979,-16.9379881452606,
-21.4488891139657));
#67171=CARTESIAN_POINT('Ctrl Pts',(-19.4593420684319,-16.9618019016887,
-21.444514398924));
#67172=CARTESIAN_POINT('Ctrl Pts',(-19.5269739887336,-16.989124238982,-21.4401396838823));
#67173=CARTESIAN_POINT('Ctrl Pts',(-19.5945855447919,-17.0164383494096,
-21.435766286085));
#67174=CARTESIAN_POINT('Ctrl Pts',(-19.6608063422521,-17.0472587627945,
-21.4313928882876));
#67175=CARTESIAN_POINT('Ctrl Pts',(-19.7252559661585,-17.0814116942643,
-21.4270194904902));
#67176=CARTESIAN_POINT('Ctrl Pts',(-19.7897074198449,-17.115565595365,-21.4226459685284));
#67177=CARTESIAN_POINT('Ctrl Pts',(-19.852387175046,-17.1530519748722,-21.4182724465665));
#67178=CARTESIAN_POINT('Ctrl Pts',(-19.9129394590442,-17.1936511290678,
-21.4138989246046));
#67179=CARTESIAN_POINT('Ctrl Pts',(-19.9735547443612,-17.2342925244489,
-21.4095208522338));
#67180=CARTESIAN_POINT('Ctrl Pts',(-20.0320377377389,-17.2780528916324,
-21.4051427798631));
#67181=CARTESIAN_POINT('Ctrl Pts',(-20.0880624200393,-17.3246696823824,
-21.4007647074923));
#67182=CARTESIAN_POINT('Ctrl Pts',(-20.1441178009626,-17.3713120167183,
-21.3963842361647));
#67183=CARTESIAN_POINT('Ctrl Pts',(-20.1977118344489,-17.420813563513,-21.3920037648371));
#67184=CARTESIAN_POINT('Ctrl Pts',(-20.2485543554084,-17.4728738713303,
-21.3876232935095));
#67185=CARTESIAN_POINT('Ctrl Pts',(-20.2994870055889,-17.5250264671557,
-21.3832350568615));
#67186=CARTESIAN_POINT('Ctrl Pts',(-20.3476580839202,-17.5797465198983,
-21.3788468202134));
#67187=CARTESIAN_POINT('Ctrl Pts',(-20.3928171932228,-17.6366998367413,
-21.3744585835654));
#67188=CARTESIAN_POINT('Ctrl Pts',(-20.4234261084619,-17.6753028843823,
-21.3714842298706));
#67189=CARTESIAN_POINT('Ctrl Pts',(-20.4526521461855,-17.7149312605343,
-21.3685098761757));
#67190=CARTESIAN_POINT('Ctrl Pts',(-20.4804290453301,-17.7554739494572,
-21.3655355224809));
#67191=CARTESIAN_POINT('Ctrl Pts',(-20.5219871745244,-17.8161314870525,
-21.361085473018));
#67192=CARTESIAN_POINT('Ctrl Pts',(-20.5604589913813,-17.8790695530753,
-21.3566354235551));
#67193=CARTESIAN_POINT('Ctrl Pts',(-20.5955899131733,-17.9439464323899,
-21.3521853740922));
#67194=CARTESIAN_POINT('Ctrl Pts',(-20.6306645420735,-18.00871935465,-21.347742455275));
#67195=CARTESIAN_POINT('Ctrl Pts',(-20.6624086883073,-18.0754245154655,
-21.3432995364577));
#67196=CARTESIAN_POINT('Ctrl Pts',(-20.6906106838733,-18.1436908810653,
-21.3388566176404));
#67197=CARTESIAN_POINT('Ctrl Pts',(-20.7187693738979,-18.2118524203273,
-21.3344205211419));
#67198=CARTESIAN_POINT('Ctrl Pts',(-20.7433965530088,-18.2815699703269,
-21.3299844246434));
#67199=CARTESIAN_POINT('Ctrl Pts',(-20.764326992868,-18.3524490830367,-21.3255483281449));
#67200=CARTESIAN_POINT('Ctrl Pts',(-20.7852384436445,-18.423263890871,-21.3211162562824));
#67201=CARTESIAN_POINT('Ctrl Pts',(-20.8024596851649,-18.4952377246083,
-21.31668418442));
#67202=CARTESIAN_POINT('Ctrl Pts',(-20.8158744003031,-18.5679583598586,
-21.3122521125575));
#67203=CARTESIAN_POINT('Ctrl Pts',(-20.829281573186,-18.6406381088439,-21.3078225325719));
#67204=CARTESIAN_POINT('Ctrl Pts',(-20.8388863850559,-18.7140633695048,
-21.3033929525863));
#67205=CARTESIAN_POINT('Ctrl Pts',(-20.8446233129547,-18.787810381534,-21.2989633726007));
#67206=CARTESIAN_POINT('Ctrl Pts',(-20.8489003385967,-18.8427906544308,
-21.2956610080746));
#67207=CARTESIAN_POINT('Ctrl Pts',(-20.8510286073718,-18.8979494671394,
-21.2923586435486));
#67208=CARTESIAN_POINT('Ctrl Pts',(-20.8509997094769,-18.9531090873175,
-21.2890562790225));
#67209=CARTESIAN_POINT('Ctrl Pts',(-20.8509997572016,-18.9530139075719,
-21.2873808207992));
#67210=CARTESIAN_POINT('Ctrl Pts',(-20.8509644636734,-19.0267054279197,
-21.2831945047056));
#67211=CARTESIAN_POINT('Ctrl Pts',(-20.8470814811288,-19.1003499721809,
-21.2791138391139));
#67212=CARTESIAN_POINT('Ctrl Pts',(-20.8222221592446,-19.3364815089262,
-21.2661204831227));
#67213=CARTESIAN_POINT('Ctrl Pts',(-20.7862490061281,-19.496756327703,-21.2574710226349));
#67214=CARTESIAN_POINT('Ctrl Pts',(-20.7290394438667,-19.6602350880456,
-21.2475108436966));
#67215=CARTESIAN_POINT('Ctrl Pts',(-20.7258400125798,-19.6691838473955,
-21.2469617469771));
#67216=CARTESIAN_POINT('Ctrl Pts',(-20.7225805821494,-19.6781103692267,
-21.2464098430158));
#67217=CARTESIAN_POINT('Origin',(-18.734,-18.952,0.));
#67218=CARTESIAN_POINT('',(-20.722580711674,-19.6781100145006,-20.4442392611068));
#67219=CARTESIAN_POINT('',(-20.7225805821175,-19.6781103693139,-20.6683680078465));
#67220=CARTESIAN_POINT('',(-20.7225805821191,-19.6781103693095,0.));
#67221=CARTESIAN_POINT('Ctrl Pts',(-20.7225805821175,-19.6781103693139,
-20.6683680078465));
#67222=CARTESIAN_POINT('Ctrl Pts',(-20.723865209165,-19.6745921928633,-20.6685904485746));
#67223=CARTESIAN_POINT('Ctrl Pts',(-20.7251405065262,-19.6710705886775,
-20.6688125801961));
#67224=CARTESIAN_POINT('Ctrl Pts',(-20.7310458544951,-19.6546273968654,
-20.6698473346312));
#67225=CARTESIAN_POINT('Ctrl Pts',(-20.7355595809394,-19.6416641653527,
-20.6706561060802));
#67226=CARTESIAN_POINT('Ctrl Pts',(-20.768858785208,-19.5429489113029,-20.6767638662585));
#67227=CARTESIAN_POINT('Ctrl Pts',(-20.7922497624033,-19.4554696483961,
-20.6818795550824));
#67228=CARTESIAN_POINT('Ctrl Pts',(-20.8373639001823,-19.2296587432863,
-20.6946257986702));
#67229=CARTESIAN_POINT('Ctrl Pts',(-20.8511051846752,-19.0901947745664,
-20.7020608620861));
#67230=CARTESIAN_POINT('Ctrl Pts',(-20.8509840406084,-18.9301095183909,
-20.7109057851118));
#67231=CARTESIAN_POINT('Ctrl Pts',(-20.8506770340003,-18.9098227212298,
-20.7120328634699));
#67232=CARTESIAN_POINT('Ctrl Pts',(-20.8483264214982,-18.8301815006497,
-20.7164921316393));
#67233=CARTESIAN_POINT('Ctrl Pts',(-20.8440773295534,-18.7709246959545,
-20.7198853747503));
#67234=CARTESIAN_POINT('Ctrl Pts',(-20.8363297185987,-18.703044686032,-20.723937924618));
#67235=CARTESIAN_POINT('Ctrl Pts',(-20.8352591867053,-18.6941651343004,
-20.7244713321321));
#67236=CARTESIAN_POINT('Ctrl Pts',(-20.8335616364937,-18.6807981145446,
-20.7252796168894));
#67237=CARTESIAN_POINT('Ctrl Pts',(-20.8329764089932,-18.6763053106714,
-20.7255521954006));
#67238=CARTESIAN_POINT('Ctrl Pts',(-20.8319046584194,-18.6682787131095,
-20.726040842706));
#67239=CARTESIAN_POINT('Ctrl Pts',(-20.8314236225146,-18.6647442395577,
-20.7262565992299));
#67240=CARTESIAN_POINT('Ctrl Pts',(-20.8303644475976,-18.6571063331617,
-20.7267241180625));
#67241=CARTESIAN_POINT('Ctrl Pts',(-20.8297832008255,-18.6530034342164,
-20.7269760486134));
#67242=CARTESIAN_POINT('Ctrl Pts',(-20.8281309523601,-18.6415821188147,
-20.7276795047986));
#67243=CARTESIAN_POINT('Ctrl Pts',(-20.8270336495137,-18.6342676521319,
-20.7281324773477));
#67244=CARTESIAN_POINT('Ctrl Pts',(-20.820538960699,-18.5924691228918,-20.7307345037716));
#67245=CARTESIAN_POINT('Ctrl Pts',(-20.8143280497843,-18.5581190996876,
-20.732925459951));
#67246=CARTESIAN_POINT('Ctrl Pts',(-20.7918958200027,-18.449470363468,-20.7399904291395));
#67247=CARTESIAN_POINT('Ctrl Pts',(-20.7725200329496,-18.3758873924989,
-20.7449760667154));
#67248=CARTESIAN_POINT('Ctrl Pts',(-20.6904215811938,-18.1207597792959,
-20.7626582812333));
#67249=CARTESIAN_POINT('Ctrl Pts',(-20.607011625039,-17.9468115910366,-20.7753362062963));
#67250=CARTESIAN_POINT('Ctrl Pts',(-20.4894885235568,-17.7686120090818,
-20.7884544750299));
#67251=CARTESIAN_POINT('Ctrl Pts',(-20.4774343679079,-17.750923919569,-20.7897596960255));
#67252=CARTESIAN_POINT('Ctrl Pts',(-20.4603097930515,-17.7265967405172,
-20.791559750663));
#67253=CARTESIAN_POINT('Ctrl Pts',(-20.455465536487,-17.7198007223895,-20.7920631596211));
#67254=CARTESIAN_POINT('Ctrl Pts',(-20.4470413638233,-17.7081290786888,
-20.7929287332018));
#67255=CARTESIAN_POINT('Ctrl Pts',(-20.4434805340322,-17.7032398597014,
-20.7932916276391));
#67256=CARTESIAN_POINT('Ctrl Pts',(-20.4360698635491,-17.6931556940307,
-20.7940407786998));
#67257=CARTESIAN_POINT('Ctrl Pts',(-20.4322170744055,-17.6879629844414,
-20.7944269154879));
#67258=CARTESIAN_POINT('Ctrl Pts',(-20.4231495398308,-17.675858236915,-20.7953279585973));
#67259=CARTESIAN_POINT('Ctrl Pts',(-20.4179160356735,-17.6689603452745,
-20.7958421240079));
#67260=CARTESIAN_POINT('Ctrl Pts',(-20.4008332352383,-17.6467293514784,
-20.7975016805812));
#67261=CARTESIAN_POINT('Ctrl Pts',(-20.3888154824816,-17.6315265031748,
-20.7986404092484));
#67262=CARTESIAN_POINT('Ctrl Pts',(-20.3265596628857,-17.5549558727395,
-20.8043990523528));
#67263=CARTESIAN_POINT('Ctrl Pts',(-20.2731076957359,-17.4962774859446,
-20.8088863626349));
#67264=CARTESIAN_POINT('Ctrl Pts',(-20.1000686770742,-17.3265342060466,
-20.8223349060607));
#67265=CARTESIAN_POINT('Ctrl Pts',(-19.9708583089203,-17.2261788962322,
-20.8309359319349));
#67266=CARTESIAN_POINT('Ctrl Pts',(-19.7791771957653,-17.1099832231012,
-20.8434651877469));
#67267=CARTESIAN_POINT('Ctrl Pts',(-19.7255935311021,-17.0805935827379,
-20.8469516357444));
#67268=CARTESIAN_POINT('Ctrl Pts',(-19.6626469889472,-17.0495313841536,
-20.8511147944165));
#67269=CARTESIAN_POINT('Ctrl Pts',(-19.654448179116,-17.0455511527494,-20.8516583326422));
#67270=CARTESIAN_POINT('Ctrl Pts',(-19.642158524247,-17.0396827165673,-20.8524753631453));
#67271=CARTESIAN_POINT('Ctrl Pts',(-19.6380868132261,-17.0377543702632,
-20.8527464286688));
#67272=CARTESIAN_POINT('Ctrl Pts',(-19.6307806650308,-17.0343227173495,
-20.8532335425438));
#67273=CARTESIAN_POINT('Ctrl Pts',(-19.6275485583818,-17.032814575116,-20.853449287818));
#67274=CARTESIAN_POINT('Ctrl Pts',(-19.6205324220565,-17.0295623222176,
-20.8539181837594));
#67275=CARTESIAN_POINT('Ctrl Pts',(-19.6167470999229,-17.0278212356431,
-20.8541715103589));
#67276=CARTESIAN_POINT('Ctrl Pts',(-19.6061407962318,-17.0229806728741,
-20.8548822451461));
#67277=CARTESIAN_POINT('Ctrl Pts',(-19.5993085431071,-17.0199062511749,
-20.8553411458966));
#67278=CARTESIAN_POINT('Ctrl Pts',(-19.5591795513974,-17.0021042886336,
-20.8580420997529));
#67279=CARTESIAN_POINT('Ctrl Pts',(-19.5255257813601,-16.9882023662435,
-20.8603297434085));
#67280=CARTESIAN_POINT('Ctrl Pts',(-19.4153870013204,-16.9459964143811,
-20.867850708044));
#67281=CARTESIAN_POINT('Ctrl Pts',(-19.3376237011844,-16.9212426779879,
-20.8732108566154));
#67282=CARTESIAN_POINT('Ctrl Pts',(-19.0810906874427,-16.8556220082492,
-20.8906948988151));
#67283=CARTESIAN_POINT('Ctrl Pts',(-18.8983629531948,-16.8334429315667,
-20.9027594792982));
#67284=CARTESIAN_POINT('Ctrl Pts',(-18.6927250276458,-16.8352847743648,
-20.9154088693627));
#67285=CARTESIAN_POINT('Ctrl Pts',(-18.6704146050536,-16.8358374525744,
-20.9167705395927));
#67286=CARTESIAN_POINT('Ctrl Pts',(-18.6396301837634,-16.8370873605794,
-20.9186352418421));
#67287=CARTESIAN_POINT('Ctrl Pts',(-18.6311460223452,-16.8374829872602,
-20.9191476686827));
#67288=CARTESIAN_POINT('Ctrl Pts',(-18.6165842214634,-16.8382498715001,
-20.920024686603));
#67289=CARTESIAN_POINT('Ctrl Pts',(-18.6105054302373,-16.8385963085047,
-20.920390051414));
#67290=CARTESIAN_POINT('Ctrl Pts',(-18.5979928579742,-16.8393635839881,
-20.9211406155645));
#67291=CARTESIAN_POINT('Ctrl Pts',(-18.591559329758,-16.8397875992643,-20.9215257112028));
#67292=CARTESIAN_POINT('Ctrl Pts',(-18.5766198067645,-16.8408407875793,
-20.9224180998122));
#67293=CARTESIAN_POINT('Ctrl Pts',(-18.5681154392479,-16.8414919897895,
-20.9229246961162));
#67294=CARTESIAN_POINT('Ctrl Pts',(-18.5410187258285,-16.8437316543733,
-20.9245345206078));
#67295=CARTESIAN_POINT('Ctrl Pts',(-18.5224430221923,-16.8455145698367,
-20.9256316433706));
#67296=CARTESIAN_POINT('Ctrl Pts',(-18.3441739464121,-16.8650070012947,
-20.936104450901));
#67297=CARTESIAN_POINT('Ctrl Pts',(-18.1869591311987,-16.9005959487609,
-20.9448516755273));
#67298=CARTESIAN_POINT('Ctrl Pts',(-17.9084942866733,-16.9979616726981,
-20.9608714191344));
#67299=CARTESIAN_POINT('Ctrl Pts',(-17.7862430511598,-17.0542454535539,
-20.9681340845894));
#67300=CARTESIAN_POINT('Ctrl Pts',(-17.6566079943566,-17.1295946355659,
-20.9769255817016));
#67301=CARTESIAN_POINT('Ctrl Pts',(-17.6431404604304,-17.1376239974544,
-20.9778531014542));
#67302=CARTESIAN_POINT('Ctrl Pts',(-17.6248246786053,-17.1488215231846,
-20.9791358277245));
#67303=CARTESIAN_POINT('Ctrl Pts',(-17.6198980247693,-17.1518613109438,
-20.9794829963443));
#67304=CARTESIAN_POINT('Ctrl Pts',(-17.6120883509842,-17.156724286518,-20.9800368289494));
#67305=CARTESIAN_POINT('Ctrl Pts',(-17.6091971209646,-17.1585343274685,
-20.9802426318032));
#67306=CARTESIAN_POINT('Ctrl Pts',(-17.6032372336692,-17.1622855671119,
-20.9806684816565));
#67307=CARTESIAN_POINT('Ctrl Pts',(-17.600169203859,-17.1642276683136,-20.9808885916277));
#67308=CARTESIAN_POINT('Ctrl Pts',(-17.5928705750823,-17.1688741358451,
-20.981414321515));
#67309=CARTESIAN_POINT('Ctrl Pts',(-17.5886445864649,-17.1715856697601,
-20.9817204144978));
#67310=CARTESIAN_POINT('Ctrl Pts',(-17.5744205112017,-17.1807839067649,
-20.9827562835207));
#67311=CARTESIAN_POINT('Ctrl Pts',(-17.564467779022,-17.1873398602394,-20.9834904712269));
#67312=CARTESIAN_POINT('Ctrl Pts',(-17.5406895091441,-17.203292332644,-20.9852661703009));
#67313=CARTESIAN_POINT('Ctrl Pts',(-17.5269190639248,-17.2127691325323,
-20.9863123277161));
#67314=CARTESIAN_POINT('Ctrl Pts',(-17.4756950857485,-17.2489227495913,
-20.9902669456693));
#67315=CARTESIAN_POINT('Ctrl Pts',(-17.4390035992435,-17.2766531241249,
-20.9932277158313));
#67316=CARTESIAN_POINT('Ctrl Pts',(-17.3454265824065,-17.3522875177858,
-21.0010643322817));
#67317=CARTESIAN_POINT('Ctrl Pts',(-17.2901100640836,-17.4020330766274,
-21.0059879963955));
#67318=CARTESIAN_POINT('Ctrl Pts',(-17.1277255407977,-17.5643153714376,
-21.0211549223784));
#67319=CARTESIAN_POINT('Ctrl Pts',(-17.030308298842,-17.6858098785556,-21.0312706877406));
#67320=CARTESIAN_POINT('Ctrl Pts',(-16.9342096445632,-17.8370933919803,
-21.0423125955737));
#67321=CARTESIAN_POINT('Ctrl Pts',(-16.9217171620446,-17.8575169908679,
-21.0437748597252));
#67322=CARTESIAN_POINT('Ctrl Pts',(-16.9046537626209,-17.8865069658841,
-21.0458116978412));
#67323=CARTESIAN_POINT('Ctrl Pts',(-16.8997915892861,-17.8948989769513,
-21.0463968450537));
#67324=CARTESIAN_POINT('Ctrl Pts',(-16.8920196577054,-17.9085282434224,
-21.0473400426544));
#67325=CARTESIAN_POINT('Ctrl Pts',(-16.8890742006779,-17.9137448847618,
-21.047699380446));
#67326=CARTESIAN_POINT('Ctrl Pts',(-16.8829819480667,-17.9246425422203,
-21.0484465936299));
#67327=CARTESIAN_POINT('Ctrl Pts',(-16.8798390665344,-17.930325683547,-21.0488343254957));
#67328=CARTESIAN_POINT('Ctrl Pts',(-16.8724722135699,-17.943792813822,-21.0497485918363));
#67329=CARTESIAN_POINT('Ctrl Pts',(-16.8682708156304,-17.9515890623656,
-21.0502743159918));
#67330=CARTESIAN_POINT('Ctrl Pts',(-16.8544957143635,-17.9775392009793,
-21.0520126536078));
#67331=CARTESIAN_POINT('Ctrl Pts',(-16.8451368942052,-17.9958062853925,
-21.0532176622835));
#67332=CARTESIAN_POINT('Ctrl Pts',(-16.7969204161315,-18.0933893498731,
-21.0595611632357));
#67333=CARTESIAN_POINT('Ctrl Pts',(-16.7627868894722,-18.1749472340003,
-21.0645331899724));
#67334=CARTESIAN_POINT('Ctrl Pts',(-16.6909636103039,-18.3820681892771,
-21.0766335480794));
#67335=CARTESIAN_POINT('Ctrl Pts',(-16.6596436015191,-18.5094347336584,
-21.0836107002132));
#67336=CARTESIAN_POINT('Ctrl Pts',(-16.634706335176,-18.6761780249987,-21.0929106682711));
#67337=CARTESIAN_POINT('Ctrl Pts',(-16.6301256108669,-18.7136221971592,
-21.0950110809277));
#67338=CARTESIAN_POINT('Ctrl Pts',(-16.6221958036023,-18.7968341192315,
-21.0997427780473));
#67339=CARTESIAN_POINT('Ctrl Pts',(-16.6193297501016,-18.8426269120661,
-21.1023893118999));
#67340=CARTESIAN_POINT('Ctrl Pts',(-16.6177244973075,-18.8960967451019,
-21.1055661122373));
#67341=CARTESIAN_POINT('Ctrl Pts',(-16.617536821783,-18.9037217596845,-21.1060211891972));
#67342=CARTESIAN_POINT('Ctrl Pts',(-16.6173018883948,-18.9159537791142,
-21.1067547501936));
#67343=CARTESIAN_POINT('Ctrl Pts',(-16.6172284559638,-18.9205602933888,
-21.1070318079103));
#67344=CARTESIAN_POINT('Ctrl Pts',(-16.6171246682075,-18.9287479991062,
-21.1075257395748));
#67345=CARTESIAN_POINT('Ctrl Pts',(-16.6170883627061,-18.9323290672215,
-21.1077422775414));
#67346=CARTESIAN_POINT('Ctrl Pts',(-16.6170304189219,-18.9399527748725,
-21.1082043602753));
#67347=CARTESIAN_POINT('Ctrl Pts',(-16.6170112736669,-18.9439953270453,
-21.1084500359427));
#67348=CARTESIAN_POINT('Ctrl Pts',(-16.6169907237168,-18.9549753220759,
-21.1091190402344));
#67349=CARTESIAN_POINT('Ctrl Pts',(-16.6170118413194,-18.9619126857155,
-21.109543598171));
#67350=CARTESIAN_POINT('Ctrl Pts',(-16.6172932041723,-18.9972620389329,
-21.1117160260678));
#67351=CARTESIAN_POINT('Ctrl Pts',(-16.6180913198089,-19.0256653586692,
-21.1134914872741));
#67352=CARTESIAN_POINT('Ctrl Pts',(-16.6221156261413,-19.109057745881,-21.1187756317686));
#67353=CARTESIAN_POINT('Ctrl Pts',(-16.6269164156029,-19.1639449947982,
-21.1223445100066));
#67354=CARTESIAN_POINT('Ctrl Pts',(-16.6514713538496,-19.357392784989,-21.135115341163));
#67355=CARTESIAN_POINT('Ctrl Pts',(-16.6828132132105,-19.4941315393559,
-21.1444672079832));
#67356=CARTESIAN_POINT('Ctrl Pts',(-16.7562372029758,-19.7124716697801,
-21.1593415142229));
#67357=CARTESIAN_POINT('Ctrl Pts',(-16.7905170766199,-19.7962397232974,
-21.1650403125865));
#67358=CARTESIAN_POINT('Ctrl Pts',(-16.8360578917058,-19.8899196901911,
-21.1713959949041));
#67359=CARTESIAN_POINT('Ctrl Pts',(-16.8421821526842,-19.9022119964556,
-21.1722297439337));
#67360=CARTESIAN_POINT('Ctrl Pts',(-16.8521965011511,-19.9218316279638,
-21.1735603356539));
#67361=CARTESIAN_POINT('Ctrl Pts',(-16.8560107186651,-19.9291970410959,
-21.1740598207493));
#67362=CARTESIAN_POINT('Ctrl Pts',(-16.8628604740812,-19.9422359684906,
-21.1749440587411));
#67363=CARTESIAN_POINT('Ctrl Pts',(-16.8658787581825,-19.9479183832198,
-21.175329414469));
#67364=CARTESIAN_POINT('Ctrl Pts',(-16.8722219962547,-19.9597302656751,
-21.176130484694));
#67365=CARTESIAN_POINT('Ctrl Pts',(-16.8755514267536,-19.96585725128,-21.17654603432));
#67366=CARTESIAN_POINT('Ctrl Pts',(-16.8842776700188,-19.9817282994689,
-21.1776225832501));
#67367=CARTESIAN_POINT('Ctrl Pts',(-16.8897212647759,-19.9914464982501,
-21.1782819047145));
#67368=CARTESIAN_POINT('Ctrl Pts',(-16.913706544352,-20.0334846631622,-21.1811350176553));
#67369=CARTESIAN_POINT('Ctrl Pts',(-16.9330236523287,-20.0653560913092,
-21.1833007414704));
#67370=CARTESIAN_POINT('Ctrl Pts',(-16.9865970614789,-20.1487008703966,
-21.1889869142468));
#67371=CARTESIAN_POINT('Ctrl Pts',(-17.0222841596487,-20.199212789821,-21.1924562191714));
#67372=CARTESIAN_POINT('Ctrl Pts',(-17.1467978282404,-20.3600185623447,
-21.2037083688439));
#67373=CARTESIAN_POINT('Ctrl Pts',(-17.244465309878,-20.4629636279903,-21.211232481966));
#67374=CARTESIAN_POINT('Ctrl Pts',(-17.4090638204192,-20.6048687831921,
-21.2232630176597));
#67375=CARTESIAN_POINT('Ctrl Pts',(-17.4690650998353,-20.6512257663225,
-21.2275443446769));
#67376=CARTESIAN_POINT('Ctrl Pts',(-17.5392393551531,-20.6996631281265,
-21.2325977268907));
#67377=CARTESIAN_POINT('Ctrl Pts',(-17.5471006958358,-20.7050115350583,
-21.2331644703743));
#67378=CARTESIAN_POINT('Ctrl Pts',(-17.5588073131143,-20.7128612063167,
-21.2340097870987));
#67379=CARTESIAN_POINT('Ctrl Pts',(-17.5626252450527,-20.7154033066165,
-21.2342856862601));
#67380=CARTESIAN_POINT('Ctrl Pts',(-17.5694383459189,-20.7199077962093,
-21.2347784625273));
#67381=CARTESIAN_POINT('Ctrl Pts',(-17.5724302594645,-20.7218750124284,
-21.2349950118591));
#67382=CARTESIAN_POINT('Ctrl Pts',(-17.5788828540481,-20.7260942552716,
-21.2354623749235));
#67383=CARTESIAN_POINT('Ctrl Pts',(-17.5823450925328,-20.7283437226215,
-21.2357133476784));
#67384=CARTESIAN_POINT('Ctrl Pts',(-17.5919287779979,-20.7345305886333,
-21.2364085628659));
#67385=CARTESIAN_POINT('Ctrl Pts',(-17.5980639170006,-20.7384465251871,
-21.2368541848435));
#67386=CARTESIAN_POINT('Ctrl Pts',(-17.6319421156355,-20.7598252261794,
-21.2393174960063));
#67387=CARTESIAN_POINT('Ctrl Pts',(-17.6600661054577,-20.7766723941025,
-21.2413718829415));
#67388=CARTESIAN_POINT('Ctrl Pts',(-17.8308836100605,-20.8736804273696,
-21.2538542178134));
#67389=CARTESIAN_POINT('Ctrl Pts',(-17.9820874314102,-20.9377247233029,
-21.2648714402771));
#67390=CARTESIAN_POINT('Ctrl Pts',(-18.2489541487524,-21.0158575328392,
-21.2830116145616));
#67391=CARTESIAN_POINT('Ctrl Pts',(-18.3611878695894,-21.0390543424456,
-21.2902911434788));
#67392=CARTESIAN_POINT('Ctrl Pts',(-18.4889224800171,-21.0548146728704,
-21.2981492569332));
#67393=CARTESIAN_POINT('Ctrl Pts',(-18.5030993886727,-21.0564185568766,
-21.2990158239945));
#67394=CARTESIAN_POINT('Ctrl Pts',(-18.525705743568,-21.0587448940237,-21.3003889799335));
#67395=CARTESIAN_POINT('Ctrl Pts',(-18.5341249893068,-21.0595603263237,
-21.3008984733819));
#67396=CARTESIAN_POINT('Ctrl Pts',(-18.5489925275914,-21.0609104050816,
-21.3017948850917));
#67397=CARTESIAN_POINT('Ctrl Pts',(-18.5554387657245,-21.0614659865855,
-21.3021824555291));
#67398=CARTESIAN_POINT('Ctrl Pts',(-18.5687870401352,-21.0625548081514,
-21.3029827754518));
#67399=CARTESIAN_POINT('Ctrl Pts',(-18.5756893555835,-21.0630837647827,
-21.3033953861626));
#67400=CARTESIAN_POINT('Ctrl Pts',(-18.5934347757626,-21.0643561583935,
-21.3044530871225));
#67401=CARTESIAN_POINT('Ctrl Pts',(-18.6042813204718,-21.0650499740904,
-21.305096617988));
#67402=CARTESIAN_POINT('Ctrl Pts',(-18.6497597959553,-21.0676075730786,
-21.3077829067901));
#67403=CARTESIAN_POINT('Ctrl Pts',(-18.6844306700201,-21.0687037816909,
-21.3098016289608));
#67404=CARTESIAN_POINT('Ctrl Pts',(-18.7749976417425,-21.0693406171065,
-21.3150108688458));
#67405=CARTESIAN_POINT('Ctrl Pts',(-18.8308771138604,-21.0675206425202,
-21.3181607867753));
#67406=CARTESIAN_POINT('Ctrl Pts',(-19.0845521969156,-21.0491845589789,
-21.332294817397));
#67407=CARTESIAN_POINT('Ctrl Pts',(-19.2794561066504,-21.0071224258054,
-21.3426052650713));
#67408=CARTESIAN_POINT('Ctrl Pts',(-19.4955714179402,-20.9275293304824,
-21.3558293489102));
#67409=CARTESIAN_POINT('Ctrl Pts',(-19.525258987734,-20.9158269089208,-21.3576899172998));
#67410=CARTESIAN_POINT('Ctrl Pts',(-19.5609542872504,-20.9008155632122,
-21.3599938570517));
#67411=CARTESIAN_POINT('Ctrl Pts',(-19.5672267492959,-20.8981419973941,
-21.3604012509739));
#67412=CARTESIAN_POINT('Ctrl Pts',(-19.5775380098296,-20.8936879531629,
-21.3610753296728));
#67413=CARTESIAN_POINT('Ctrl Pts',(-19.5815844043926,-20.8919250393001,
-21.3613409679403));
#67414=CARTESIAN_POINT('Ctrl Pts',(-19.5888753552902,-20.8887213867386,
-21.3618216678));
#67415=CARTESIAN_POINT('Ctrl Pts',(-19.5921218304316,-20.887285128067,-21.3620364532172));
#67416=CARTESIAN_POINT('Ctrl Pts',(-19.5984334106447,-20.8844738455263,
-21.3624554896874));
#67417=CARTESIAN_POINT('Ctrl Pts',(-19.6014988122479,-20.8830997114248,
-21.3626596782347));
#67418=CARTESIAN_POINT('Ctrl Pts',(-19.6105424044381,-20.8790198424555,
-21.3632640343987));
#67419=CARTESIAN_POINT('Ctrl Pts',(-19.6165112337142,-20.8762936313696,
-21.3636654434041));
#67420=CARTESIAN_POINT('Ctrl Pts',(-19.6448669640108,-20.8631827205932,
-21.3655841187029));
#67421=CARTESIAN_POINT('Ctrl Pts',(-19.6670827966634,-20.8524353154302,
-21.3671222453472));
#67422=CARTESIAN_POINT('Ctrl Pts',(-19.7292807475042,-20.8209922084031,
-21.3715174049684));
#67423=CARTESIAN_POINT('Ctrl Pts',(-19.7687964036886,-20.7994067013962,
-21.374415197408));
#67424=CARTESIAN_POINT('Ctrl Pts',(-19.88952039456,-20.728372134586,-21.3835369426157));
#67425=CARTESIAN_POINT('Ctrl Pts',(-19.968107776952,-20.6747021716754,-21.3898620877258));
#67426=CARTESIAN_POINT('Ctrl Pts',(-20.160632426997,-20.5232656827976,-21.4060183990992));
#67427=CARTESIAN_POINT('Ctrl Pts',(-20.2682886293656,-20.4183322888617,
-21.4156928769252));
#67428=CARTESIAN_POINT('Ctrl Pts',(-20.3729857267611,-20.2920053876034,
-21.4257089935953));
#67429=CARTESIAN_POINT('Ctrl Pts',(-20.3818931560424,-20.2810360465027,
-21.4265671086272));
#67430=CARTESIAN_POINT('Ctrl Pts',(-20.3959063430243,-20.263421558129,-21.4279269323577));
#67431=CARTESIAN_POINT('Ctrl Pts',(-20.4010835075936,-20.2568340039992,
-21.4284315172946));
#67432=CARTESIAN_POINT('Ctrl Pts',(-20.4101513952445,-20.2451537298734,
-21.4293192798389));
#67433=CARTESIAN_POINT('Ctrl Pts',(-20.4140583306603,-20.2400737850971,
-21.4297031032954));
#67434=CARTESIAN_POINT('Ctrl Pts',(-20.4220971023071,-20.2295226717649,
-21.430495646683));
#67435=CARTESIAN_POINT('Ctrl Pts',(-20.4262255532588,-20.2240490093937,
-21.4309042295636));
#67436=CARTESIAN_POINT('Ctrl Pts',(-20.4367657948163,-20.2099322157558,
-21.4319514664971));
#67437=CARTESIAN_POINT('Ctrl Pts',(-20.4431384531545,-20.2012600073221,
-21.432588579356));
#67438=CARTESIAN_POINT('Ctrl Pts',(-20.4695463826491,-20.1647425511917,
-21.4352459081674));
#67439=CARTESIAN_POINT('Ctrl Pts',(-20.488970148204,-20.1364600957453,-21.437242430499));
#67440=CARTESIAN_POINT('Ctrl Pts',(-20.5378432110347,-20.0614537507977,
-21.442391173593));
#67441=CARTESIAN_POINT('Ctrl Pts',(-20.5661674189159,-20.0140269094543,
-21.4455035225487));
#67442=CARTESIAN_POINT('Ctrl Pts',(-20.6274484735311,-19.9016515664535,
-21.4526164833822));
#67443=CARTESIAN_POINT('Ctrl Pts',(-20.658973887806,-19.8360030591184,-21.4565792730157));
#67444=CARTESIAN_POINT('Ctrl Pts',(-20.6995927811212,-19.7388860102984,
-21.4622948261543));
#67445=CARTESIAN_POINT('Ctrl Pts',(-20.7114372793834,-19.7086282580148,
-21.4640561413387));
#67446=CARTESIAN_POINT('Ctrl Pts',(-20.722580582091,-19.6781103693865,-21.465822579505));
#67447=CARTESIAN_POINT('Ctrl Pts',(-20.7225805821494,-19.6781103692267,
-21.2464098430158));
#67448=CARTESIAN_POINT('Ctrl Pts',(-20.7151809012897,-19.698375692923,-21.2451568900026));
#67449=CARTESIAN_POINT('Ctrl Pts',(-20.7074719860344,-19.7185264049827,
-21.2438894700321));
#67450=CARTESIAN_POINT('Ctrl Pts',(-20.6968058209637,-19.7451791787207,
-21.2421798140781));
#67451=CARTESIAN_POINT('Ctrl Pts',(-20.6941216461761,-19.7517893655548,
-21.2417530485997));
#67452=CARTESIAN_POINT('Ctrl Pts',(-20.6898485633233,-19.7621617588142,
-21.2410788630868));
#67453=CARTESIAN_POINT('Ctrl Pts',(-20.6882820649243,-19.7659332209493,
-21.2408327803363));
#67454=CARTESIAN_POINT('Ctrl Pts',(-20.6853241227265,-19.7729969202685,
-21.2403700669868));
#67455=CARTESIAN_POINT('Ctrl Pts',(-20.6839352503089,-19.7762901758043,
-21.2401535926792));
#67456=CARTESIAN_POINT('Ctrl Pts',(-20.6807339855021,-19.783827558518,-21.239656439768));
#67457=CARTESIAN_POINT('Ctrl Pts',(-20.6789160539789,-19.7880692791049,
-21.2393754270876));
#67458=CARTESIAN_POINT('Ctrl Pts',(-20.6732460556527,-19.801180334003,-21.23850306994));
#67459=CARTESIAN_POINT('Ctrl Pts',(-20.6693471421221,-19.8100290993669,
-21.2379089766039));
#67460=CARTESIAN_POINT('Ctrl Pts',(-20.6276874059676,-19.9028491342297,
-21.2316233024324));
#67461=CARTESIAN_POINT('Ctrl Pts',(-20.5845514899138,-19.9842893332979,
-21.2256463578304));
#67462=CARTESIAN_POINT('Ctrl Pts',(-20.4721083710498,-20.1667509646173,
-21.2115516109801));
#67463=CARTESIAN_POINT('Ctrl Pts',(-20.3990542360701,-20.2651025885536,
-21.2034109595741));
#67464=CARTESIAN_POINT('Ctrl Pts',(-20.2756220774325,-20.4042926086402,
-21.1913749560756));
#67465=CARTESIAN_POINT('Ctrl Pts',(-20.2311926486573,-20.4500546900007,
-21.1873152381914));
#67466=CARTESIAN_POINT('Ctrl Pts',(-20.1664053107302,-20.511018717677,-21.1817683175493));
#67467=CARTESIAN_POINT('Ctrl Pts',(-20.1477410408678,-20.5279634166997,
-21.1802101097512));
#67468=CARTESIAN_POINT('Ctrl Pts',(-20.1189668361614,-20.553163937167,-21.1778667360507));
#67469=CARTESIAN_POINT('Ctrl Pts',(-20.1090763545244,-20.5616658417592,
-21.1770714691907));
#67470=CARTESIAN_POINT('Ctrl Pts',(-20.0907048659911,-20.5771651522004,
-21.1756127710069));
#67471=CARTESIAN_POINT('Ctrl Pts',(-20.0822467551121,-20.584188886067,-21.1749482736233));
#67472=CARTESIAN_POINT('Ctrl Pts',(-20.0684444358686,-20.5954700245966,
-21.1738751989208));
#67473=CARTESIAN_POINT('Ctrl Pts',(-20.0631337397865,-20.5997679380398,
-21.1734649829231));
#67474=CARTESIAN_POINT('Ctrl Pts',(-20.0530398016817,-20.6078563483877,
-21.1726902874773));
#67475=CARTESIAN_POINT('Ctrl Pts',(-20.0482608031583,-20.6116520079229,
-21.1723256027671));
#67476=CARTESIAN_POINT('Ctrl Pts',(-20.0371069785972,-20.6204324038952,
-21.1714792774759));
#67477=CARTESIAN_POINT('Ctrl Pts',(-20.0307198245265,-20.6254013814665,
-21.1709982678441));
#67478=CARTESIAN_POINT('Ctrl Pts',(-20.0141841566172,-20.6381140161988,
-21.1697621944453));
#67479=CARTESIAN_POINT('Ctrl Pts',(-20.0039937205729,-20.6458027957396,
-21.1690092928549));
#67480=CARTESIAN_POINT('Ctrl Pts',(-19.9390512959285,-20.693886866537,-21.1642655842235));
#67481=CARTESIAN_POINT('Ctrl Pts',(-19.8824450058645,-20.731717368187,-21.1603753219429));
#67482=CARTESIAN_POINT('Ctrl Pts',(-19.6842207853306,-20.8507889829137,
-21.1474096945091));
#67483=CARTESIAN_POINT('Ctrl Pts',(-19.5350931339249,-20.9183587656678,
-21.1387753113413));
#67484=CARTESIAN_POINT('Ctrl Pts',(-19.3268970384958,-20.9850358507186,
-21.126700253472));
#67485=CARTESIAN_POINT('Ctrl Pts',(-19.2734664663781,-20.9998615054935,
-21.123594526353));
#67486=CARTESIAN_POINT('Ctrl Pts',(-19.1917461770392,-21.0191167450673,
-21.1187518383991));
#67487=CARTESIAN_POINT('Ctrl Pts',(-19.1638446024887,-21.0250983182965,
-21.117082298086));
#67488=CARTESIAN_POINT('Ctrl Pts',(-19.129008203159,-21.0318331249412,-21.1149682959755));
#67489=CARTESIAN_POINT('Ctrl Pts',(-19.1221778031881,-21.0331187612011,
-21.1145523991981));
#67490=CARTESIAN_POINT('Ctrl Pts',(-19.1113601054842,-21.0350997893233,
-21.1138913254639));
#67491=CARTESIAN_POINT('Ctrl Pts',(-19.1073768621791,-21.0358174343373,
-21.113647395275));
#67492=CARTESIAN_POINT('Ctrl Pts',(-19.0998621341073,-21.0371490947439,
-21.1131861925066));
#67493=CARTESIAN_POINT('Ctrl Pts',(-19.0963311398356,-21.037765565178,-21.1129690612158));
#67494=CARTESIAN_POINT('Ctrl Pts',(-19.0882556979009,-21.0391543184373,
-21.1124715243904));
#67495=CARTESIAN_POINT('Ctrl Pts',(-19.0837102896108,-21.0399207266753,
-21.1121907899535));
#67496=CARTESIAN_POINT('Ctrl Pts',(-19.0716369458633,-21.0419159008968,
-21.1114433573562));
#67497=CARTESIAN_POINT('Ctrl Pts',(-19.0641048904745,-21.0431188242895,
-21.1109752549015));
#67498=CARTESIAN_POINT('Ctrl Pts',(-19.0113293099853,-21.051255227184,-21.1076834758471));
#67499=CARTESIAN_POINT('Ctrl Pts',(-18.9658812712963,-21.0567599492808,
-21.1047878632221));
#67500=CARTESIAN_POINT('Ctrl Pts',(-18.9096436732841,-21.0617280930136,
-21.1011583933981));
#67501=CARTESIAN_POINT('Ctrl Pts',(-18.8989859729359,-21.0625882944636,
-21.1004685066869));
#67502=CARTESIAN_POINT('Ctrl Pts',(-18.7360005561771,-21.0745010916135,
-21.0898909620382));
#67503=CARTESIAN_POINT('Ctrl Pts',(-18.5829201314274,-21.0691191483902,
-21.0796342248313));
#67504=CARTESIAN_POINT('Ctrl Pts',(-18.3398835153214,-21.0340603373794,
-21.0636972639725));
#67505=CARTESIAN_POINT('Ctrl Pts',(-18.2489842435714,-21.0147813028083,
-21.0578076430166));
#67506=CARTESIAN_POINT('Ctrl Pts',(-18.1393414552467,-20.9838746727492,
-21.0508125005824));
#67507=CARTESIAN_POINT('Ctrl Pts',(-18.1191357823133,-20.9778517998307,
-21.0495277076858));
#67508=CARTESIAN_POINT('Ctrl Pts',(-18.0904777832314,-20.9688411919096,
-21.0477110701582));
#67509=CARTESIAN_POINT('Ctrl Pts',(-18.0819497443941,-20.9661002221531,
-21.0471711860068));
#67510=CARTESIAN_POINT('Ctrl Pts',(-18.0672475774973,-20.9612716787602,
-21.0462415917969));
#67511=CARTESIAN_POINT('Ctrl Pts',(-18.061065269426,-20.9592095859284,-21.0458510489854));
#67512=CARTESIAN_POINT('Ctrl Pts',(-18.0492323639408,-20.9552019361616,
-21.0451041963304));
#67513=CARTESIAN_POINT('Ctrl Pts',(-18.0435802983861,-20.9532609398044,
-21.0447477402189));
#67514=CARTESIAN_POINT('Ctrl Pts',(-18.0288741174594,-20.9481409195988,
-21.043820969016));
#67515=CARTESIAN_POINT('Ctrl Pts',(-18.0198331983671,-20.9449241995567,
-21.0432519085));
#67516=CARTESIAN_POINT('Ctrl Pts',(-17.9889239525977,-20.9336894763137,
-21.0413085124323));
#67517=CARTESIAN_POINT('Ctrl Pts',(-17.9671657534014,-20.9253719361747,
-21.0399441529836));
#67518=CARTESIAN_POINT('Ctrl Pts',(-17.7867624565159,-20.8529743856351,
-21.0286518996669));
#67519=CARTESIAN_POINT('Ctrl Pts',(-17.6362869280282,-20.7702396597499,
-21.0194319214345));
#67520=CARTESIAN_POINT('Ctrl Pts',(-17.4242275491654,-20.6176266887034,
-21.0052256167648));
#67521=CARTESIAN_POINT('Ctrl Pts',(-17.3544997997982,-20.5603509426405,
-21.000300137549));
#67522=CARTESIAN_POINT('Ctrl Pts',(-17.2604303378236,-20.4724512888722,
-20.9929553840031));
#67523=CARTESIAN_POINT('Ctrl Pts',(-17.2329484304121,-20.445326298497,-20.9907140073888));
#67524=CARTESIAN_POINT('Ctrl Pts',(-17.2009536051128,-20.4119711469122,
-20.9879643324888));
#67525=CARTESIAN_POINT('Ctrl Pts',(-17.1957115255254,-20.4064468240535,
-20.9875091327688));
#67526=CARTESIAN_POINT('Ctrl Pts',(-17.1876306650577,-20.3978383207474,
-20.9867998873983));
#67527=CARTESIAN_POINT('Ctrl Pts',(-17.1847709836745,-20.3947737258723,
-20.9865474158765));
#67528=CARTESIAN_POINT('Ctrl Pts',(-17.1794976182552,-20.3890887368434,
-20.9860790539247));
#67529=CARTESIAN_POINT('Ctrl Pts',(-17.177081440136,-20.3864707350773,-20.9858633588662));
#67530=CARTESIAN_POINT('Ctrl Pts',(-17.1716505172992,-20.3805562813599,
-20.985376054872));
#67531=CARTESIAN_POINT('Ctrl Pts',(-17.1686396098713,-20.3772563991359,
-20.985104163261));
#67532=CARTESIAN_POINT('Ctrl Pts',(-17.1598311659693,-20.3675409753861,
-20.9843037118207));
#67533=CARTESIAN_POINT('Ctrl Pts',(-17.1540625473198,-20.3610995035121,
-20.9837730572173));
#67534=CARTESIAN_POINT('Ctrl Pts',(-17.1140943616616,-20.3159154402178,
-20.9800522807053));
#67535=CARTESIAN_POINT('Ctrl Pts',(-17.0812867997021,-20.2759704416452,
-20.9767710271767));
#67536=CARTESIAN_POINT('Ctrl Pts',(-17.0366100744695,-20.2173232628266,
-20.9720114015117));
#67537=CARTESIAN_POINT('Ctrl Pts',(-17.0235191220997,-20.1995698929873,
-20.9705777308999));
#67538=CARTESIAN_POINT('Ctrl Pts',(-16.9840342976884,-20.144232382046,-20.966137766717));
#67539=CARTESIAN_POINT('Ctrl Pts',(-16.9585843969024,-20.1059918777097,
-20.9631098909174));
#67540=CARTESIAN_POINT('Ctrl Pts',(-16.8768042599706,-19.9739940599948,
-20.9528524498352));
#67541=CARTESIAN_POINT('Ctrl Pts',(-16.8264948390657,-19.8767028731446,
-20.9456214661846));
#67542=CARTESIAN_POINT('Ctrl Pts',(-16.7624917060153,-19.725225034177,-20.9350516013849));
#67543=CARTESIAN_POINT('Ctrl Pts',(-16.7430436419927,-19.6736754860697,
-20.9315643118513));
#67544=CARTESIAN_POINT('Ctrl Pts',(-16.7147840953464,-19.5888923770621,
-20.9260094054404));
#67545=CARTESIAN_POINT('Ctrl Pts',(-16.7047327990432,-19.5561023197927,
-20.9239033881697));
#67546=CARTESIAN_POINT('Ctrl Pts',(-16.6925670008698,-19.5126755570457,
-20.9211678392338));
#67547=CARTESIAN_POINT('Ctrl Pts',(-16.6897316436486,-19.5022478207212,
-20.9205149824574));
#67548=CARTESIAN_POINT('Ctrl Pts',(-16.685217618378,-19.4851297404333,-20.9194496972804));
#67549=CARTESIAN_POINT('Ctrl Pts',(-16.6834916088089,-19.4784521885083,
-20.9190357400471));
#67550=CARTESIAN_POINT('Ctrl Pts',(-16.6802131660186,-19.4655078583839,
-20.9182363370981));
#67551=CARTESIAN_POINT('Ctrl Pts',(-16.6786567087105,-19.4592421871588,
-20.9178507651476));
#67552=CARTESIAN_POINT('Ctrl Pts',(-16.67512833542,-19.4447554572578,-20.9169624231352));
#67553=CARTESIAN_POINT('Ctrl Pts',(-16.6731769453728,-19.4365294754173,
-20.9164603192327));
#67554=CARTESIAN_POINT('Ctrl Pts',(-16.6680598806704,-19.4143684912192,
-20.9151137450957));
#67555=CARTESIAN_POINT('Ctrl Pts',(-16.6649859002001,-19.400412609178,-20.9142722168645));
#67556=CARTESIAN_POINT('Ctrl Pts',(-16.6380607690271,-19.271996305939,-20.9065856210845));
#67557=CARTESIAN_POINT('Ctrl Pts',(-16.6235870997623,-19.1557683937764,
-20.9000577587314));
#67558=CARTESIAN_POINT('Ctrl Pts',(-16.612097379801,-18.8761836513789,-20.8847397841375));
#67559=CARTESIAN_POINT('Ctrl Pts',(-16.6242138937639,-18.7132333547738,
-20.8761329405072));
#67560=CARTESIAN_POINT('Ctrl Pts',(-16.6609684104183,-18.5215660670561,
-20.8649248914188));
#67561=CARTESIAN_POINT('Ctrl Pts',(-16.6677801148839,-18.4899735165662,
-20.863039780627));
#67562=CARTESIAN_POINT('Ctrl Pts',(-16.6769960023837,-18.4515244600164,
-20.8606855787975));
#67563=CARTESIAN_POINT('Ctrl Pts',(-16.6787161943862,-18.4445064657664,
-20.8602534085993));
#67564=CARTESIAN_POINT('Ctrl Pts',(-16.6814702302107,-18.4335143144678,
-20.8595724420682));
#67565=CARTESIAN_POINT('Ctrl Pts',(-16.682479785303,-18.4295340489524,-20.859325025088));
#67566=CARTESIAN_POINT('Ctrl Pts',(-16.6843892282124,-18.4220967587648,
-20.8588611041058));
#67567=CARTESIAN_POINT('Ctrl Pts',(-16.6852862879052,-18.4186390658179,
-20.858644764284));
#67568=CARTESIAN_POINT('Ctrl Pts',(-16.6873549502471,-18.4107476831028,
-20.8581495268807));
#67569=CARTESIAN_POINT('Ctrl Pts',(-16.6885322068715,-18.4063155338617,
-20.8578703058359));
#67570=CARTESIAN_POINT('Ctrl Pts',(-16.6921982200937,-18.3926922466135,
-20.8570088212555));
#67571=CARTESIAN_POINT('Ctrl Pts',(-16.6947345554561,-18.3835141951356,
-20.8564239044982));
#67572=CARTESIAN_POINT('Ctrl Pts',(-16.7185357292232,-18.2995959243037,
-20.8510361990448));
#67573=CARTESIAN_POINT('Ctrl Pts',(-16.743836590417,-18.2260701042058,-20.8460290686741));
#67574=CARTESIAN_POINT('Ctrl Pts',(-16.788529564351,-18.1162333045789,-20.8382678938088));
#67575=CARTESIAN_POINT('Ctrl Pts',(-16.8050356844214,-18.0788117456707,
-20.8355711291447));
#67576=CARTESIAN_POINT('Ctrl Pts',(-16.8696063712948,-17.94320199509,-20.8256493319105));
#67577=CARTESIAN_POINT('Ctrl Pts',(-16.9241745769758,-17.8482915134168,
-20.8184220279744));
#67578=CARTESIAN_POINT('Ctrl Pts',(-17.0168587405443,-17.7125883932035,
-20.8078598389365));
#67579=CARTESIAN_POINT('Ctrl Pts',(-17.0496457258955,-17.668385286558,-20.8043765462533));
#67580=CARTESIAN_POINT('Ctrl Pts',(-17.1055891224957,-17.5988034141636,
-20.7988271578512));
#67581=CARTESIAN_POINT('Ctrl Pts',(-17.1277043407155,-17.5726242511841,
-20.7967227675539));
#67582=CARTESIAN_POINT('Ctrl Pts',(-17.1576169442291,-17.5389104083168,
-20.7939889082263));
#67583=CARTESIAN_POINT('Ctrl Pts',(-17.1648493857497,-17.5308835061051,
-20.7933361569086));
#67584=CARTESIAN_POINT('Ctrl Pts',(-17.1767991672402,-17.5178235323663,
-20.7922709472738));
#67585=CARTESIAN_POINT('Ctrl Pts',(-17.1814801501911,-17.5127575980527,
-20.7918569613977));
#67586=CARTESIAN_POINT('Ctrl Pts',(-17.190591411671,-17.5029932264992,-20.7910574359211));
#67587=CARTESIAN_POINT('Ctrl Pts',(-17.1950185883894,-17.4982920113303,
-20.7906717704168));
#67588=CARTESIAN_POINT('Ctrl Pts',(-17.2052937529954,-17.4874803708258,
-20.7897831160845));
#67589=CARTESIAN_POINT('Ctrl Pts',(-17.2111570117524,-17.4813845607437,
-20.7892807942162));
#67590=CARTESIAN_POINT('Ctrl Pts',(-17.2270312020111,-17.4650774993905,
-20.7879334180775));
#67591=CARTESIAN_POINT('Ctrl Pts',(-17.2371094313686,-17.4549321587139,
-20.7870913100847));
#67592=CARTESIAN_POINT('Ctrl Pts',(-17.3310036155552,-17.3623089324332,
-20.779364792049));
#67593=CARTESIAN_POINT('Ctrl Pts',(-17.4214570547904,-17.286841479805,-20.7728014692284));
#67594=CARTESIAN_POINT('Ctrl Pts',(-17.6516594578399,-17.1252524985302,
-20.7574079964102));
#67595=CARTESIAN_POINT('Ctrl Pts',(-17.7960292751888,-17.0470942151458,
-20.7487611914907));
#67596=CARTESIAN_POINT('Ctrl Pts',(-17.9767199868582,-16.9748361343166,
-20.7375685113015));
#67597=CARTESIAN_POINT('Ctrl Pts',(-18.0057509713667,-16.9639599868621,
-20.7357583226344));
#67598=CARTESIAN_POINT('Ctrl Pts',(-18.041742500261,-16.9513702367761,-20.7334874885538));
#67599=CARTESIAN_POINT('Ctrl Pts',(-18.0484882638105,-16.9490487894883,
-20.7330607358659));
#67600=CARTESIAN_POINT('Ctrl Pts',(-18.0591164680737,-16.9454512417125,
-20.7323863937624));
#67601=CARTESIAN_POINT('Ctrl Pts',(-18.062991161965,-16.9441521871218,-20.732140138974));
#67602=CARTESIAN_POINT('Ctrl Pts',(-18.0702630837045,-16.9417375565125,
-20.7316771606436));
#67603=CARTESIAN_POINT('Ctrl Pts',(-18.0736593846302,-16.9406193655189,
-20.7314605938004));
#67604=CARTESIAN_POINT('Ctrl Pts',(-18.0814483199326,-16.9380768066054,
-20.7309631694134));
#67605=CARTESIAN_POINT('Ctrl Pts',(-18.0858427797469,-16.9366582074118,
-20.7306819776656));
#67606=CARTESIAN_POINT('Ctrl Pts',(-18.0994689304275,-16.9323086530672,
-20.7298084506056));
#67607=CARTESIAN_POINT('Ctrl Pts',(-18.1087159687357,-16.9294267164841,
-20.729213355607));
#67608=CARTESIAN_POINT('Ctrl Pts',(-18.2199628802434,-16.8955912489628,
-20.7220292534648));
#67609=CARTESIAN_POINT('Ctrl Pts',(-18.324128948869,-16.8723241983385,-20.7150599223007));
#67610=CARTESIAN_POINT('Ctrl Pts',(-18.5378458842779,-16.8412703940283,
-20.700813451564));
#67611=CARTESIAN_POINT('Ctrl Pts',(-18.6471661833861,-16.8339540624244,
-20.6935567741784));
#67612=CARTESIAN_POINT('Ctrl Pts',(-18.8191791912484,-16.8357877355927,
-20.6824361753263));
#67613=CARTESIAN_POINT('Ctrl Pts',(-18.8817359967659,-16.8392328358894,
-20.6784511901261));
#67614=CARTESIAN_POINT('Ctrl Pts',(-18.9688258376729,-16.8479169160879,
-20.6729961074588));
#67615=CARTESIAN_POINT('Ctrl Pts',(-18.9935540026917,-16.8508239959902,
-20.6714575304749));
#67616=CARTESIAN_POINT('Ctrl Pts',(-19.036759637992,-16.8566777328146,-20.6687868523993));
#67617=CARTESIAN_POINT('Ctrl Pts',(-19.0552596515311,-16.8594343323808,
-20.6676489700601));
#67618=CARTESIAN_POINT('Ctrl Pts',(-19.0821456222421,-16.8638054513975,
-20.6660031193632));
#67619=CARTESIAN_POINT('Ctrl Pts',(-19.090561795757,-16.8652260457255,-20.6654890348276));
#67620=CARTESIAN_POINT('Ctrl Pts',(-19.1053189666751,-16.8678088429808,
-20.6645895244084));
#67621=CARTESIAN_POINT('Ctrl Pts',(-19.1116636326348,-16.8689491758432,
-20.6642034090808));
#67622=CARTESIAN_POINT('Ctrl Pts',(-19.1239854232061,-16.8712219301125,
-20.6634547123123));
#67623=CARTESIAN_POINT('Ctrl Pts',(-19.1299630637734,-16.8723511691265,
-20.6630920337509));
#67624=CARTESIAN_POINT('Ctrl Pts',(-19.1442606325555,-16.8751160100363,
-20.6622258044872));
#67625=CARTESIAN_POINT('Ctrl Pts',(-19.1525758062836,-16.8767758694626,
-20.6617230309353));
#67626=CARTESIAN_POINT('Ctrl Pts',(-19.1826603860175,-16.882969475897,-20.6599074474704));
#67627=CARTESIAN_POINT('Ctrl Pts',(-19.2043684754828,-16.8877962784277,
-20.6586039909661));
#67628=CARTESIAN_POINT('Ctrl Pts',(-19.4052514603699,-16.9357963450666,
-20.6465932891083));
#67629=CARTESIAN_POINT('Ctrl Pts',(-19.5781410126775,-17.001849293089,-20.6367286530683));
#67630=CARTESIAN_POINT('Ctrl Pts',(-19.8115637456355,-17.1279644304358,
-20.6222693001478));
#67631=CARTESIAN_POINT('Ctrl Pts',(-19.8805505657211,-17.1705205217267,
-20.6178176188594));
#67632=CARTESIAN_POINT('Ctrl Pts',(-19.9766422664143,-17.2376943237939,
-20.6111128236623));
#67633=CARTESIAN_POINT('Ctrl Pts',(-20.0058197364711,-17.2592277303693,
-20.609004110606));
#67634=CARTESIAN_POINT('Ctrl Pts',(-20.040330275753,-17.2860929914317,-20.6064014951247));
#67635=CARTESIAN_POINT('Ctrl Pts',(-20.0462081769648,-17.2907189740851,
-20.6059543080364));
#67636=CARTESIAN_POINT('Ctrl Pts',(-20.0553184657506,-17.2979674015733,
-20.6052548840553));
#67637=CARTESIAN_POINT('Ctrl Pts',(-20.0585679101481,-17.3005684466764,
-20.605004152083));
#67638=CARTESIAN_POINT('Ctrl Pts',(-20.064586644847,-17.3054153852174,-20.6045373436736));
#67639=CARTESIAN_POINT('Ctrl Pts',(-20.0673579396073,-17.3076586980289,
-20.6043214519178));
#67640=CARTESIAN_POINT('Ctrl Pts',(-20.0736189984585,-17.3127531466337,
-20.6038315428823));
#67641=CARTESIAN_POINT('Ctrl Pts',(-20.0771053160298,-17.3156084159083,
-20.6035572294908));
#67642=CARTESIAN_POINT('Ctrl Pts',(-20.087394471296,-17.3240901923961,-20.6027432103989));
#67643=CARTESIAN_POINT('Ctrl Pts',(-20.0941711619113,-17.3297480649717,
-20.6022013047546));
#67644=CARTESIAN_POINT('Ctrl Pts',(-20.1437896734811,-17.371704121525,-20.5981920727157));
#67645=CARTESIAN_POINT('Ctrl Pts',(-20.1852038922591,-17.4096485278185,
-20.5946172570416));
#67646=CARTESIAN_POINT('Ctrl Pts',(-20.2694067173499,-17.4931928310492,
-20.5869375741964));
#67647=CARTESIAN_POINT('Ctrl Pts',(-20.3117850996791,-17.5391356368496,
-20.5828223138073));
#67648=CARTESIAN_POINT('Ctrl Pts',(-20.4227519187064,-17.6706641931095,
-20.5714554048852));
#67649=CARTESIAN_POINT('Ctrl Pts',(-20.4868273101149,-17.7598152940171,
-20.564205795166));
#67650=CARTESIAN_POINT('Ctrl Pts',(-20.5724489149629,-17.90087597484,-20.5535967989467));
#67651=CARTESIAN_POINT('Ctrl Pts',(-20.599318236279,-17.9493311416735,-20.5500891540958));
#67652=CARTESIAN_POINT('Ctrl Pts',(-20.6397608396946,-18.029530453112,-20.5445055773609));
#67653=CARTESIAN_POINT('Ctrl Pts',(-20.6545119754037,-18.060647985304,-20.5423907557199));
#67654=CARTESIAN_POINT('Ctrl Pts',(-20.6728942822845,-18.1020028838744,
-20.5396455710918));
#67655=CARTESIAN_POINT('Ctrl Pts',(-20.6772145069152,-18.1119264780837,
-20.5389916811012));
#67656=CARTESIAN_POINT('Ctrl Pts',(-20.6841645653466,-18.1282313471316,
-20.537925111408));
#67657=CARTESIAN_POINT('Ctrl Pts',(-20.6868395931637,-18.1345930325052,
-20.5375108962547));
#67658=CARTESIAN_POINT('Ctrl Pts',(-20.6919565598858,-18.1469305737922,
-20.5367112718804));
#67659=CARTESIAN_POINT('Ctrl Pts',(-20.6944023640957,-18.1529047342856,
-20.536325734962));
#67660=CARTESIAN_POINT('Ctrl Pts',(-20.6999852466446,-18.1667214793585,
-20.5354378681961));
#67661=CARTESIAN_POINT('Ctrl Pts',(-20.7031028042766,-18.1745718719074,
-20.5349362018097));
#67662=CARTESIAN_POINT('Ctrl Pts',(-20.7113578715634,-18.1957273899532,
-20.5335916742474));
#67663=CARTESIAN_POINT('Ctrl Pts',(-20.7164081052022,-18.209066266619,-20.5327517402014));
#67664=CARTESIAN_POINT('Ctrl Pts',(-20.7714922872059,-18.3591188841948,
-20.5233872254654));
#67665=CARTESIAN_POINT('Ctrl Pts',(-20.8074336418282,-18.5005981030119,
-20.5153747188882));
#67666=CARTESIAN_POINT('Ctrl Pts',(-20.8435716231846,-18.7468873152343,
-20.5018390224732));
#67667=CARTESIAN_POINT('Ctrl Pts',(-20.8510665767245,-18.8500662004454,
-20.496275824337));
#67668=CARTESIAN_POINT('Ctrl Pts',(-20.8509605931098,-19.0134280306006,
-20.4871374269587));
#67669=CARTESIAN_POINT('Ctrl Pts',(-20.8483662197824,-19.0734481143259,
-20.4837076978117));
#67670=CARTESIAN_POINT('Ctrl Pts',(-20.8424571655091,-19.1422045950063,
-20.4796144560487));
#67671=CARTESIAN_POINT('Ctrl Pts',(-20.8416326176233,-19.151133496576,-20.4790796927553));
#67672=CARTESIAN_POINT('Ctrl Pts',(-20.8403055945935,-19.1645707348717,
-20.4782697314217));
#67673=CARTESIAN_POINT('Ctrl Pts',(-20.8398453005765,-19.1690832658228,
-20.477996845725));
#67674=CARTESIAN_POINT('Ctrl Pts',(-20.8389970512125,-19.1771424971639,
-20.4775078488365));
#67675=CARTESIAN_POINT('Ctrl Pts',(-20.8386146293109,-19.1806897275217,
-20.4772920515391));
#67676=CARTESIAN_POINT('Ctrl Pts',(-20.8377689774517,-19.1883519337853,
-20.4768246768379));
#67677=CARTESIAN_POINT('Ctrl Pts',(-20.8373026472245,-19.1924664645893,
-20.4765729324308));
#67678=CARTESIAN_POINT('Ctrl Pts',(-20.8359714184113,-19.2039119845512,
-20.4758705576885));
#67679=CARTESIAN_POINT('Ctrl Pts',(-20.8350802524445,-19.211239774869,-20.4754184877748));
#67680=CARTESIAN_POINT('Ctrl Pts',(-20.8297855240793,-19.2529550296279,
-20.4728319418377));
#67681=CARTESIAN_POINT('Ctrl Pts',(-20.8245763695238,-19.2872327764827,
-20.4706561388139));
#67682=CARTESIAN_POINT('Ctrl Pts',(-20.805407201064,-19.3954149280918,-20.4636610476318));
#67683=CARTESIAN_POINT('Ctrl Pts',(-20.788350364743,-19.4687084470379,-20.4587324323691));
#67684=CARTESIAN_POINT('Ctrl Pts',(-20.7540340641799,-19.5871935736654,
-20.4505956310275));
#67685=CARTESIAN_POINT('Ctrl Pts',(-20.7390724262502,-19.6329445370197,
-20.4474103621586));
#67686=CARTESIAN_POINT('Ctrl Pts',(-20.7225807116741,-19.6781100145004,
-20.4442392611068));
#67687=CARTESIAN_POINT('Origin',(-18.734,-18.952,0.));
#67688=CARTESIAN_POINT('',(-20.7225805821918,-19.6781103691105,-19.6425236185391));
#67689=CARTESIAN_POINT('',(-20.7227693935251,-19.6781792853784,-19.8664843272136));
#67690=CARTESIAN_POINT('',(-20.7225805821191,-19.6781103693095,0.));
#67691=CARTESIAN_POINT('',(-20.8479201338006,-18.951171742175,-19.9109991854362));
#67692=CARTESIAN_POINT('Ctrl Pts',(-20.7227693935251,-19.6781792853784,
-19.8664843272136));
#67693=CARTESIAN_POINT('Ctrl Pts',(-20.8048847772777,-19.4459845977201,
-19.8813041251349));
#67694=CARTESIAN_POINT('Ctrl Pts',(-20.846952464507,-19.1984404792794,-19.8961239230562));
#67695=CARTESIAN_POINT('Ctrl Pts',(-20.847823891442,-18.9511685861153,-19.9109437209775));
#67696=CARTESIAN_POINT('Ctrl Pts',(-20.8509998750795,-18.9512727356193,
-19.9127740399324));
#67697=CARTESIAN_POINT('Ctrl Pts',(-20.8509329970543,-18.7565969413839,
-19.9239834015842));
#67698=CARTESIAN_POINT('Ctrl Pts',(-20.8240164173847,-18.5628627648932,
-19.9342647202721));
#67699=CARTESIAN_POINT('Ctrl Pts',(-20.7539265921552,-18.3151986713921,
-19.9484106374171));
#67700=CARTESIAN_POINT('Ctrl Pts',(-20.7341848163476,-18.2556675204103,
-19.9519023759823));
#67701=CARTESIAN_POINT('Ctrl Pts',(-20.7008062966819,-18.1682154893869,
-19.9572865832378));
#67702=CARTESIAN_POINT('Ctrl Pts',(-20.689148933844,-18.1395730264876,-19.9590923501055));
#67703=CARTESIAN_POINT('Ctrl Pts',(-20.6740381863279,-18.1046561236404,
-19.9613582347434));
#67704=CARTESIAN_POINT('Ctrl Pts',(-20.6711741824253,-18.0981288195114,
-19.9617846298524));
#67705=CARTESIAN_POINT('Ctrl Pts',(-20.6666170550983,-18.0878836845935,
-19.9624585183398));
#67706=CARTESIAN_POINT('Ctrl Pts',(-20.6649460104447,-18.0841560092348,
-19.9627046797831));
#67707=CARTESIAN_POINT('Ctrl Pts',(-20.66179207534,-18.0771745887545,-19.9631675666607));
#67708=CARTESIAN_POINT('Ctrl Pts',(-20.6603117271982,-18.0739197560113,
-19.9633841359097));
#67709=CARTESIAN_POINT('Ctrl Pts',(-20.6568999800879,-18.0664685173876,
-19.9638816696385));
#67710=CARTESIAN_POINT('Ctrl Pts',(-20.6549630923311,-18.062274684474,-19.9641629690023));
#67711=CARTESIAN_POINT('Ctrl Pts',(-20.6489187126931,-18.0492988762204,
-19.9650371755357));
#67712=CARTESIAN_POINT('Ctrl Pts',(-20.6447646758537,-18.0405388980323,
-19.9656328485742));
#67713=CARTESIAN_POINT('Ctrl Pts',(-20.5974983407664,-17.9426075312916,
-19.9723513825971));
#67714=CARTESIAN_POINT('Ctrl Pts',(-20.5482438232996,-17.8565485333077,
-19.9788036086315));
#67715=CARTESIAN_POINT('Ctrl Pts',(-20.3994705247197,-17.6343296035303,
-19.9964201072025));
#67716=CARTESIAN_POINT('Ctrl Pts',(-20.2894060373859,-17.5060483292051,
-20.0076072383412));
#67717=CARTESIAN_POINT('Ctrl Pts',(-20.1424171177537,-17.3711730409822,
-20.0201341058102));
#67718=CARTESIAN_POINT('Ctrl Pts',(-20.1190845959435,-17.3506900764286,
-20.0220635731716));
#67719=CARTESIAN_POINT('Ctrl Pts',(-20.0837111244639,-17.3209885883243,
-20.0249032042272));
#67720=CARTESIAN_POINT('Ctrl Pts',(-20.0720088310794,-17.3113748962161,
-20.0258292017461));
#67721=CARTESIAN_POINT('Ctrl Pts',(-20.0531030042032,-17.2961801840757,
-20.0273041307332));
#67722=CARTESIAN_POINT('Ctrl Pts',(-20.0459650155932,-17.2905187932341,
-20.0278562767433));
#67723=CARTESIAN_POINT('Ctrl Pts',(-20.032281594028,-17.279809154674,-20.0289058492431));
#67724=CARTESIAN_POINT('Ctrl Pts',(-20.0257427224932,-17.2747528320202,
-20.0294035922447));
#67725=CARTESIAN_POINT('Ctrl Pts',(-20.01421400205,-17.2659454119496,-20.030274561818));
#67726=CARTESIAN_POINT('Ctrl Pts',(-20.0092368956509,-17.2621778714327,
-20.0306484353059));
#67727=CARTESIAN_POINT('Ctrl Pts',(-19.9993815351404,-17.2547859586397,
-20.0313845884839));
#67728=CARTESIAN_POINT('Ctrl Pts',(-19.9945041966061,-17.2511604710649,
-20.0317469096997));
#67729=CARTESIAN_POINT('Ctrl Pts',(-19.9828033277665,-17.2425408021907,
-20.0326114133704));
#67730=CARTESIAN_POINT('Ctrl Pts',(-19.9759653205673,-17.2375663774657,
-20.0331128257484));
#67731=CARTESIAN_POINT('Ctrl Pts',(-19.9511593222597,-17.2197471280602,
-20.0349182820432));
#67732=CARTESIAN_POINT('Ctrl Pts',(-19.9330199963934,-17.2071424326034,
-20.0362131104266));
#67733=CARTESIAN_POINT('Ctrl Pts',(-19.7605250822278,-17.091239235717,-20.0483000397543));
#67734=CARTESIAN_POINT('Ctrl Pts',(-19.5934087661266,-17.0083933158489,
-20.0582339598155));
#67735=CARTESIAN_POINT('Ctrl Pts',(-19.34184897396,-16.9225623314705,-20.0727242238513));
#67736=CARTESIAN_POINT('Ctrl Pts',(-19.2646841100287,-16.9010319360953,
-20.0771269185047));
#67737=CARTESIAN_POINT('Ctrl Pts',(-19.1513181956848,-16.8762276177192,
-20.0837651271762));
#67738=CARTESIAN_POINT('Ctrl Pts',(-19.1159556306609,-16.8694306715644,
-20.0858595222651));
#67739=CARTESIAN_POINT('Ctrl Pts',(-19.0730752307487,-16.8623175572817,
-20.0884462581942));
#67740=CARTESIAN_POINT('Ctrl Pts',(-19.0657047598637,-16.8611349464801,
-20.0888925479951));
#67741=CARTESIAN_POINT('Ctrl Pts',(-19.0542183933179,-16.8593541919355,
-20.0895908735595));
#67742=CARTESIAN_POINT('Ctrl Pts',(-19.0501066449248,-16.8587291418022,
-20.0898414120969));
#67743=CARTESIAN_POINT('Ctrl Pts',(-19.042466088925,-16.857590682762,-20.0903080542773));
#67744=CARTESIAN_POINT('Ctrl Pts',(-19.0389378164005,-16.857074072032,-20.0905239744579));
#67745=CARTESIAN_POINT('Ctrl Pts',(-19.0309431720641,-16.8559241182523,
-20.09101419882));
#67746=CARTESIAN_POINT('Ctrl Pts',(-19.0264760935226,-16.8552961383814,
-20.0912888006934));
#67747=CARTESIAN_POINT('Ctrl Pts',(-19.0149359627932,-16.8537114286811,
-20.09199990662));
#67748=CARTESIAN_POINT('Ctrl Pts',(-19.0078600843968,-16.8527761923558,
-20.0924375781615));
#67749=CARTESIAN_POINT('Ctrl Pts',(-18.9643547654437,-16.8472496894368,
-20.0951381493054));
#67750=CARTESIAN_POINT('Ctrl Pts',(-18.9278180434111,-16.843571348409,-20.0974473660306));
#67751=CARTESIAN_POINT('Ctrl Pts',(-18.7213427963177,-16.8281961996241,
-20.1106611846892));
#67752=CARTESIAN_POINT('Ctrl Pts',(-18.5505747211863,-16.8360933337509,
-20.1221541195018));
#67753=CARTESIAN_POINT('Ctrl Pts',(-18.2884304756434,-16.8802193876888,
-20.1394304840613));
#67754=CARTESIAN_POINT('Ctrl Pts',(-18.1954371985372,-16.9024240731352,
-20.1454976502872));
#67755=CARTESIAN_POINT('Ctrl Pts',(-18.0838147822577,-16.9372031578587,
-20.1526793179893));
#67756=CARTESIAN_POINT('Ctrl Pts',(-18.063476885015,-16.9438799992159,-20.1539839864423));
#67757=CARTESIAN_POINT('Ctrl Pts',(-18.0347244211766,-16.953804844348,-20.1558235435656));
#67758=CARTESIAN_POINT('Ctrl Pts',(-18.0262244632704,-16.9567997572317,
-20.1563667515203));
#67759=CARTESIAN_POINT('Ctrl Pts',(-18.0116019152073,-16.9620571349953,
-20.1573002549157));
#67760=CARTESIAN_POINT('Ctrl Pts',(-18.00547023807,-16.9642937877145,-20.1576914019878));
#67761=CARTESIAN_POINT('Ctrl Pts',(-17.993755266139,-16.9686285503661,-20.1584381771184));
#67762=CARTESIAN_POINT('Ctrl Pts',(-17.9881703117364,-16.9707219653826,
-20.1587939573603));
#67763=CARTESIAN_POINT('Ctrl Pts',(-17.9736826109668,-16.9762223474794,
-20.1597163031347));
#67764=CARTESIAN_POINT('Ctrl Pts',(-17.9647938323402,-16.9796659156173,
-20.1602816379677));
#67765=CARTESIAN_POINT('Ctrl Pts',(-17.9346252640623,-16.9915883753866,
-20.1621987222366));
#67766=CARTESIAN_POINT('Ctrl Pts',(-17.9134594912385,-17.0003527367573,
-20.1635408625983));
#67767=CARTESIAN_POINT('Ctrl Pts',(-17.7303956665289,-17.0796608672349,
-20.1751347597013));
#67768=CARTESIAN_POINT('Ctrl Pts',(-17.5777740492076,-17.169859802721,-20.1846244359568));
#67769=CARTESIAN_POINT('Ctrl Pts',(-17.3699313704298,-17.3307533985968,
-20.1989284464757));
#67770=CARTESIAN_POINT('Ctrl Pts',(-17.3050419795286,-17.387646972506,-20.2036512495653));
#67771=CARTESIAN_POINT('Ctrl Pts',(-17.217082933855,-17.474817791539,-20.2107230866526));
#67772=CARTESIAN_POINT('Ctrl Pts',(-17.1910710207122,-17.5020088158801,
-20.2129089615281));
#67773=CARTESIAN_POINT('Ctrl Pts',(-17.1607204334145,-17.535476945143,-20.2155971437152));
#67774=CARTESIAN_POINT('Ctrl Pts',(-17.1556717596129,-17.5411044966881,
-20.216049077638));
#67775=CARTESIAN_POINT('Ctrl Pts',(-17.1478789038328,-17.5498850477863,
-20.2167543284615));
#67776=CARTESIAN_POINT('Ctrl Pts',(-17.1451136752056,-17.5530194007364,
-20.2170060997183));
#67777=CARTESIAN_POINT('Ctrl Pts',(-17.1400078814819,-17.5588414203773,
-20.21747384555));
#67778=CARTESIAN_POINT('Ctrl Pts',(-17.137664814137,-17.5615268159126,-20.2176896291192));
#67779=CARTESIAN_POINT('Ctrl Pts',(-17.1323895818204,-17.5676036810643,
-20.2181780108206));
#67780=CARTESIAN_POINT('Ctrl Pts',(-17.1294614194031,-17.5709985365596,
-20.218450897087));
#67781=CARTESIAN_POINT('Ctrl Pts',(-17.1208693984005,-17.581024176285,-20.2192568622714));
#67782=CARTESIAN_POINT('Ctrl Pts',(-17.1152357822721,-17.5876805914954,
-20.2197920781554));
#67783=CARTESIAN_POINT('Ctrl Pts',(-17.0754246202606,-17.6353132956759,
-20.2236215820678));
#67784=CARTESIAN_POINT('Ctrl Pts',(-17.0427688019964,-17.6775306336755,
-20.2270129847817));
#67785=CARTESIAN_POINT('Ctrl Pts',(-17.0014775411127,-17.7352967883276,
-20.2316021017822));
#67786=CARTESIAN_POINT('Ctrl Pts',(-16.9913899387585,-17.7497891508251,
-20.2327493452099));
#67787=CARTESIAN_POINT('Ctrl Pts',(-16.9543067499844,-17.8045122534429,
-20.2370618079783));
#67788=CARTESIAN_POINT('Ctrl Pts',(-16.9285139369384,-17.8455389606142,
-20.2402556476629));
#67789=CARTESIAN_POINT('Ctrl Pts',(-16.8491461703863,-17.9819589767084,
-20.2506813367774));
#67790=CARTESIAN_POINT('Ctrl Pts',(-16.8015464442096,-18.0806331045793,
-20.2579141275912));
#67791=CARTESIAN_POINT('Ctrl Pts',(-16.7417568791854,-18.2338826545686,
-20.2684877683439));
#67792=CARTESIAN_POINT('Ctrl Pts',(-16.7237400994398,-18.285981135755,-20.2719769974339));
#67793=CARTESIAN_POINT('Ctrl Pts',(-16.6978381947743,-18.3715597840864,
-20.2775346885533));
#67794=CARTESIAN_POINT('Ctrl Pts',(-16.6886998489945,-18.4046306092406,
-20.2796415923459));
#67795=CARTESIAN_POINT('Ctrl Pts',(-16.6777441326697,-18.448395364119,-20.2823781553355));
#67796=CARTESIAN_POINT('Ctrl Pts',(-16.6751997356609,-18.4589003147906,
-20.2830311571577));
#67797=CARTESIAN_POINT('Ctrl Pts',(-16.6711634649893,-18.4761407653388,
-20.2840966490657));
#67798=CARTESIAN_POINT('Ctrl Pts',(-16.6696238863996,-18.4828647905609,
-20.2845106686239));
#67799=CARTESIAN_POINT('Ctrl Pts',(-16.6667069045328,-18.4958970013511,
-20.2853101715274));
#67800=CARTESIAN_POINT('Ctrl Pts',(-16.6653254436708,-18.5022041914769,
-20.2856957812267));
#67801=CARTESIAN_POINT('Ctrl Pts',(-16.6622017631382,-18.5167844867839,
-20.286584181432));
#67802=CARTESIAN_POINT('Ctrl Pts',(-16.6604801968111,-18.5250619410805,
-20.2870863059102));
#67803=CARTESIAN_POINT('Ctrl Pts',(-16.6559824485151,-18.5473566521787,
-20.2884328726699));
#67804=CARTESIAN_POINT('Ctrl Pts',(-16.6532984925475,-18.5613922235672,
-20.2892743737397));
#67805=CARTESIAN_POINT('Ctrl Pts',(-16.6299804196924,-18.6903996668701,
-20.2969545228158));
#67806=CARTESIAN_POINT('Ctrl Pts',(-16.6187513229764,-18.806874455848,-20.3034766474817));
#67807=CARTESIAN_POINT('Ctrl Pts',(-16.615014097604,-19.086361850776,-20.3187785307505));
#67808=CARTESIAN_POINT('Ctrl Pts',(-16.6315963082219,-19.2487174594628,
-20.3273754006275));
#67809=CARTESIAN_POINT('Ctrl Pts',(-16.6736061947993,-19.439368188625,-20.3385839925853));
#67810=CARTESIAN_POINT('Ctrl Pts',(-16.6813498347196,-19.4710158185405,
-20.3404840399642));
#67811=CARTESIAN_POINT('Ctrl Pts',(-16.6917037687518,-19.5094653211933,
-20.342854886854));
#67812=CARTESIAN_POINT('Ctrl Pts',(-16.693623332179,-19.5164506448447,-20.3432881531509));
#67813=CARTESIAN_POINT('Ctrl Pts',(-16.6966882472585,-19.5273839760889,
-20.3439704835333));
#67814=CARTESIAN_POINT('Ctrl Pts',(-16.697809331024,-19.5313388099488,-20.3442181595012));
#67815=CARTESIAN_POINT('Ctrl Pts',(-16.6999260225975,-19.5387237950756,
-20.3446823072514));
#67816=CARTESIAN_POINT('Ctrl Pts',(-16.7009187949994,-19.5421547004578,
-20.3448986132719));
#67817=CARTESIAN_POINT('Ctrl Pts',(-16.7032043731675,-19.5499791775736,
-20.345393446038));
#67818=CARTESIAN_POINT('Ctrl Pts',(-16.7045027522856,-19.5543710612096,
-20.3456722941024));
#67819=CARTESIAN_POINT('Ctrl Pts',(-16.7085358505881,-19.567852316147,-20.3465315437817));
#67820=CARTESIAN_POINT('Ctrl Pts',(-16.711317413698,-19.5769273903545,-20.3471145792903));
#67821=CARTESIAN_POINT('Ctrl Pts',(-16.7367684491466,-19.6580131647515,
-20.3523635292386));
#67822=CARTESIAN_POINT('Ctrl Pts',(-16.7632115404834,-19.72877460799,-20.3572224496216));
#67823=CARTESIAN_POINT('Ctrl Pts',(-16.8474928283607,-19.9221143500789,
-20.3710143398489));
#67824=CARTESIAN_POINT('Ctrl Pts',(-16.9134063328808,-20.0407945341658,
-20.3800670204478));
#67825=CARTESIAN_POINT('Ctrl Pts',(-17.0412031255139,-20.2264476862477,
-20.394673558666));
#67826=CARTESIAN_POINT('Ctrl Pts',(-17.0968741233894,-20.2972139712001,
-20.400373149202));
#67827=CARTESIAN_POINT('Ctrl Pts',(-17.1707155237133,-20.3796765933551,
-20.4071678726449));
#67828=CARTESIAN_POINT('Ctrl Pts',(-17.1847720441322,-20.3949177376972,
-20.4084309937528));
#67829=CARTESIAN_POINT('Ctrl Pts',(-17.2051779457729,-20.4164013404719,
-20.4102225718888));
#67830=CARTESIAN_POINT('Ctrl Pts',(-17.2113459827121,-20.4228136887047,
-20.4107587695586));
#67831=CARTESIAN_POINT('Ctrl Pts',(-17.2220941535637,-20.43384750951,-20.4116840183791));
#67832=CARTESIAN_POINT('Ctrl Pts',(-17.2266554701769,-20.4384870668149,
-20.4120738816011));
#67833=CARTESIAN_POINT('Ctrl Pts',(-17.2354564878018,-20.4473568838949,
-20.4128208134854));
#67834=CARTESIAN_POINT('Ctrl Pts',(-17.2396928872848,-20.451590318116,-20.4131780218039));
#67835=CARTESIAN_POINT('Ctrl Pts',(-17.250814654177,-20.462610371447,-20.4141097738007));
#67836=CARTESIAN_POINT('Ctrl Pts',(-17.2577286957619,-20.4693679531944,
-20.4146830356762));
#67837=CARTESIAN_POINT('Ctrl Pts',(-17.2817679450944,-20.4925433654805,
-20.4166559486511));
#67838=CARTESIAN_POINT('Ctrl Pts',(-17.2991230571168,-20.508720921618,-20.4180452046877));
#67839=CARTESIAN_POINT('Ctrl Pts',(-17.4372537298969,-20.6332062567327,
-20.4288424935057));
#67840=CARTESIAN_POINT('Ctrl Pts',(-17.5698440812476,-20.7275994337756,
-20.4376243940364));
#67841=CARTESIAN_POINT('Ctrl Pts',(-17.8260924463474,-20.8688692918437,
-20.4535207488873));
#67842=CARTESIAN_POINT('Ctrl Pts',(-17.9458112407303,-20.9211197571371,
-20.4606106172316));
#67843=CARTESIAN_POINT('Ctrl Pts',(-18.0808438911388,-20.965757066104,-20.4690034223024));
#67844=CARTESIAN_POINT('Ctrl Pts',(-18.0921660941425,-20.9693942714539,
-20.469710147926));
#67845=CARTESIAN_POINT('Ctrl Pts',(-18.1083101749773,-20.9744308251401,
-20.4707229111744));
#67846=CARTESIAN_POINT('Ctrl Pts',(-18.1131075513589,-20.975908783926,-20.4710244962193));
#67847=CARTESIAN_POINT('Ctrl Pts',(-18.1213859719733,-20.9784269669529,
-20.4715460767364));
#67848=CARTESIAN_POINT('Ctrl Pts',(-18.1248645571478,-20.9794753295272,
-20.4717655975527));
#67849=CARTESIAN_POINT('Ctrl Pts',(-18.1316161515226,-20.9814911548301,
-20.4721923771178));
#67850=CARTESIAN_POINT('Ctrl Pts',(-18.1348888083142,-20.9824596593024,
-20.4723995676264));
#67851=CARTESIAN_POINT('Ctrl Pts',(-18.1437281282218,-20.9850523218094,
-20.4729600179989));
#67852=CARTESIAN_POINT('Ctrl Pts',(-18.1492990979716,-20.9866615146446,
-20.4733141354594));
#67853=CARTESIAN_POINT('Ctrl Pts',(-18.1700201228114,-20.9925547226728,
-20.4746343977901));
#67854=CARTESIAN_POINT('Ctrl Pts',(-18.1852107811283,-20.9966924555437,
-20.4756084985981));
#67855=CARTESIAN_POINT('Ctrl Pts',(-18.3278347717561,-21.0338375366539,
-20.4848031192346));
#67856=CARTESIAN_POINT('Ctrl Pts',(-18.4580291706067,-21.0550577051422,
-20.4935418434554));
#67857=CARTESIAN_POINT('Ctrl Pts',(-18.748286193705,-21.0749386024076,-20.5127600440346));
#67858=CARTESIAN_POINT('Ctrl Pts',(-18.9079848879175,-21.0678496762759,
-20.5231322867377));
#67859=CARTESIAN_POINT('Ctrl Pts',(-19.0864170712931,-21.0395689391876,
-20.5342281393122));
#67860=CARTESIAN_POINT('Ctrl Pts',(-19.1073845519363,-21.0359207989438,
-20.5355251823464));
#67861=CARTESIAN_POINT('Ctrl Pts',(-19.1371281121068,-21.0302823604703,
-20.5373559650473));
#67862=CARTESIAN_POINT('Ctrl Pts',(-19.1459514913827,-21.0285514241788,
-20.5378979157303));
#67863=CARTESIAN_POINT('Ctrl Pts',(-19.1611568397871,-21.0254677686635,
-20.5388299521332));
#67864=CARTESIAN_POINT('Ctrl Pts',(-19.167544024576,-21.024141677998,-20.5392208822398));
#67865=CARTESIAN_POINT('Ctrl Pts',(-19.179763757998,-21.0215456751046,-20.5399677152005));
#67866=CARTESIAN_POINT('Ctrl Pts',(-19.1855972553064,-21.0202805780194,
-20.5403237679751));
#67867=CARTESIAN_POINT('Ctrl Pts',(-19.2007565735772,-21.0169258186646,
-20.5412478413821));
#67868=CARTESIAN_POINT('Ctrl Pts',(-19.2100738002333,-21.0147976335184,
-20.5418146221666));
#67869=CARTESIAN_POINT('Ctrl Pts',(-19.2418171196734,-21.0073204857516,
-20.5437418553954));
#67870=CARTESIAN_POINT('Ctrl Pts',(-19.2641705933201,-21.0016681998754,
-20.5450925586066));
#67871=CARTESIAN_POINT('Ctrl Pts',(-19.4549978446067,-20.9500848969666,
-20.5565785128637));
#67872=CARTESIAN_POINT('Ctrl Pts',(-19.6172811142733,-20.8838391131288,
-20.5659714918151));
#67873=CARTESIAN_POINT('Ctrl Pts',(-19.8460095525323,-20.7555518136834,
-20.5802387771242));
#67874=CARTESIAN_POINT('Ctrl Pts',(-19.919680919093,-20.7079962178389,-20.5850331460968));
#67875=CARTESIAN_POINT('Ctrl Pts',(-20.0207562854745,-20.6334843026501,
-20.592201479975));
#67876=CARTESIAN_POINT('Ctrl Pts',(-20.0507102079952,-20.6101329930742,
-20.5944071623543));
#67877=CARTESIAN_POINT('Ctrl Pts',(-20.0858688111806,-20.5811707038233,
-20.5971173035553));
#67878=CARTESIAN_POINT('Ctrl Pts',(-20.0916937761353,-20.576319571742,-20.5975704278403));
#67879=CARTESIAN_POINT('Ctrl Pts',(-20.1006932791636,-20.5687424002123,
-20.598277141533));
#67880=CARTESIAN_POINT('Ctrl Pts',(-20.1038860686648,-20.5660380002148,
-20.5985291750483));
#67881=CARTESIAN_POINT('Ctrl Pts',(-20.1097830087991,-20.561012992622,-20.5989971462403));
#67882=CARTESIAN_POINT('Ctrl Pts',(-20.1124893257759,-20.5586950164464,
-20.5992128912466));
#67883=CARTESIAN_POINT('Ctrl Pts',(-20.1185827341293,-20.5534492488169,
-20.599700855679));
#67884=CARTESIAN_POINT('Ctrl Pts',(-20.1219663773731,-20.5505175565551,
-20.5999733611393));
#67885=CARTESIAN_POINT('Ctrl Pts',(-20.1318927170447,-20.5418617939693,
-20.600777268036));
#67886=CARTESIAN_POINT('Ctrl Pts',(-20.1384093920862,-20.5361082115079,
-20.601310790974));
#67887=CARTESIAN_POINT('Ctrl Pts',(-20.184271689178,-20.4951108945783,-20.6051053299702));
#67888=CARTESIAN_POINT('Ctrl Pts',(-20.2223182614543,-20.4584484552833,
-20.6084615483248));
#67889=CARTESIAN_POINT('Ctrl Pts',(-20.2724921822122,-20.4063424455187,
-20.6131349579266));
#67890=CARTESIAN_POINT('Ctrl Pts',(-20.285838299166,-20.392093053928,-20.6144037498945));
#67891=CARTESIAN_POINT('Ctrl Pts',(-20.3975957567918,-20.2694140259198,
-20.6252362741466));
#67892=CARTESIAN_POINT('Ctrl Pts',(-20.4847189654111,-20.1512159401151,
-20.6350415699039));
#67893=CARTESIAN_POINT('Ctrl Pts',(-20.5902290846866,-19.9717611426943,
-20.648490670156));
#67894=CARTESIAN_POINT('Ctrl Pts',(-20.6191743324805,-19.9172036395424,
-20.6524167790985));
#67895=CARTESIAN_POINT('Ctrl Pts',(-20.6616864867386,-19.8278420644759,
-20.6585827761446));
#67896=CARTESIAN_POINT('Ctrl Pts',(-20.6767885703725,-19.7938119504006,
-20.6608724366706));
#67897=CARTESIAN_POINT('Ctrl Pts',(-20.6952311444707,-19.7491105817123,
-20.663807008012));
#67898=CARTESIAN_POINT('Ctrl Pts',(-20.6993949321712,-19.7387881859354,
-20.6644796971704));
#67899=CARTESIAN_POINT('Ctrl Pts',(-20.7060328946612,-19.7219505308917,
-20.6655690589631));
#67900=CARTESIAN_POINT('Ctrl Pts',(-20.7085566075863,-19.7154551479231,
-20.6659873958385));
#67901=CARTESIAN_POINT('Ctrl Pts',(-20.7133473731806,-19.7029422902167,
-20.6667896842573));
#67902=CARTESIAN_POINT('Ctrl Pts',(-20.7156191670391,-19.6969267247085,
-20.6671737914042));
#67903=CARTESIAN_POINT('Ctrl Pts',(-20.7194496029756,-19.6866424461285,
-20.6678277834673));
#67904=CARTESIAN_POINT('Ctrl Pts',(-20.7210219595117,-19.6823789306509,
-20.6680981231762));
#67905=CARTESIAN_POINT('Ctrl Pts',(-20.7225805821175,-19.6781103693139,
-20.6683680078465));
#67906=CARTESIAN_POINT('',(-20.8509992561137,-18.9502252848438,-19.6896814721675));
#67907=CARTESIAN_POINT('Ctrl Pts',(-20.7225807116741,-19.6781100145004,
-20.4442392611068));
#67908=CARTESIAN_POINT('Ctrl Pts',(-20.6728905732413,-19.8141952479699,
-20.4346846178026));
#67909=CARTESIAN_POINT('Ctrl Pts',(-20.6093080329127,-19.9449670995714,
-20.4252946123284));
#67910=CARTESIAN_POINT('Ctrl Pts',(-20.5215596583061,-20.0863590344177,
-20.4150699495229));
#67911=CARTESIAN_POINT('Ctrl Pts',(-20.5100907474605,-20.1042333354495,
-20.4137750968991));
#67912=CARTESIAN_POINT('Ctrl Pts',(-20.4937578065146,-20.1288647531108,
-20.4119869716777));
#67913=CARTESIAN_POINT('Ctrl Pts',(-20.4891202532205,-20.1357698613022,
-20.4114852708096));
#67914=CARTESIAN_POINT('Ctrl Pts',(-20.4810444557183,-20.1476425736561,
-20.4106218506718));
#67915=CARTESIAN_POINT('Ctrl Pts',(-20.4776254479406,-20.1526230851792,
-20.4102594099103));
#67916=CARTESIAN_POINT('Ctrl Pts',(-20.4705005740399,-20.1629073531736,
-20.4095104707037));
#67917=CARTESIAN_POINT('Ctrl Pts',(-20.4667916145951,-20.1682088979423,
-20.4091240952779));
#67918=CARTESIAN_POINT('Ctrl Pts',(-20.4580471986295,-20.1805868654808,
-20.4082212470825));
#67919=CARTESIAN_POINT('Ctrl Pts',(-20.452992360912,-20.187649503576,-20.4077055242836));
#67920=CARTESIAN_POINT('Ctrl Pts',(-20.4364321378702,-20.2104892116244,
-20.4060356905465));
#67921=CARTESIAN_POINT('Ctrl Pts',(-20.424751694462,-20.2261385424026,-20.4048883601294));
#67922=CARTESIAN_POINT('Ctrl Pts',(-20.3638543915206,-20.3054157388934,
-20.3990559106396));
#67923=CARTESIAN_POINT('Ctrl Pts',(-20.3112537829685,-20.3663663031307,
-20.3945074155572));
#67924=CARTESIAN_POINT('Ctrl Pts',(-20.1384828639412,-20.5449025565689,
-20.3807325628625));
#67925=CARTESIAN_POINT('Ctrl Pts',(-20.0077162827823,-20.6512792951468,
-20.371890691937));
#67926=CARTESIAN_POINT('Ctrl Pts',(-19.8645508543518,-20.7418451960285,
-20.3623780550102));
#67927=CARTESIAN_POINT('Ctrl Pts',(-19.8633371225165,-20.7426112709669,
-20.3622974162171));
#67928=CARTESIAN_POINT('Ctrl Pts',(-19.8165508761117,-20.7720750013025,
-20.3591892579398));
#67929=CARTESIAN_POINT('Ctrl Pts',(-19.769904612416,-20.7990219267759,-20.3561000848259));
#67930=CARTESIAN_POINT('Ctrl Pts',(-19.7145581433667,-20.8282385500187,
-20.3523862632687));
#67931=CARTESIAN_POINT('Ctrl Pts',(-19.7068048655429,-20.8322702084328,
-20.3518649282507));
#67932=CARTESIAN_POINT('Ctrl Pts',(-19.6950330482054,-20.8382991851899,
-20.3510714194898));
#67933=CARTESIAN_POINT('Ctrl Pts',(-19.6910326447661,-20.8403319760547,
-20.3508014210781));
#67934=CARTESIAN_POINT('Ctrl Pts',(-19.6838431722597,-20.8439565671958,
-20.3503155183131));
#67935=CARTESIAN_POINT('Ctrl Pts',(-19.6806565215616,-20.8455530449225,
-20.350099911411));
#67936=CARTESIAN_POINT('Ctrl Pts',(-19.6737267196445,-20.8490029357433,
-20.3496305209935));
#67937=CARTESIAN_POINT('Ctrl Pts',(-19.6699821599284,-20.8508532964483,
-20.3493765573496));
#67938=CARTESIAN_POINT('Ctrl Pts',(-19.659456669546,-20.8560157310239,-20.3486618363524));
#67939=CARTESIAN_POINT('Ctrl Pts',(-19.6526635481287,-20.859302606456,-20.3481995577124));
#67940=CARTESIAN_POINT('Ctrl Pts',(-19.6121125286872,-20.8786564651601,
-20.3454347298672));
#67941=CARTESIAN_POINT('Ctrl Pts',(-19.5779535986707,-20.8938621666274,
-20.3430840466224));
#67942=CARTESIAN_POINT('Ctrl Pts',(-19.4646015911746,-20.94076467045,-20.3352549237691));
#67943=CARTESIAN_POINT('Ctrl Pts',(-19.383896804573,-20.9685802419175,-20.3296386863144));
#67944=CARTESIAN_POINT('Ctrl Pts',(-19.1303458250446,-21.0391635321525,
-20.3122516409712));
#67945=CARTESIAN_POINT('Ctrl Pts',(-18.9535833238402,-21.0650899657821,
-20.3005607163423));
#67946=CARTESIAN_POINT('Ctrl Pts',(-18.7528410334991,-21.0690389430811,
-20.2882045749222));
#67947=CARTESIAN_POINT('Ctrl Pts',(-18.7300383420336,-21.0691190897398,
-20.2868128418573));
#67948=CARTESIAN_POINT('Ctrl Pts',(-18.6977240144483,-21.0687105576463,
-20.2848566525503));
#67949=CARTESIAN_POINT('Ctrl Pts',(-18.688210745538,-21.0685261351512,-20.2842827259889));
#67950=CARTESIAN_POINT('Ctrl Pts',(-18.6727398202443,-21.0681218597937,
-20.2833525042173));
#67951=CARTESIAN_POINT('Ctrl Pts',(-18.666781357925,-21.0679409704449,-20.2829949931335));
#67952=CARTESIAN_POINT('Ctrl Pts',(-18.6542980888031,-21.0675092152436,
-20.2822475400265));
#67953=CARTESIAN_POINT('Ctrl Pts',(-18.6477735098318,-21.0672533248515,
-20.2818577594565));
#67954=CARTESIAN_POINT('Ctrl Pts',(-18.6322316958416,-21.0665717536709,
-20.2809313521401));
#67955=CARTESIAN_POINT('Ctrl Pts',(-18.6232157471918,-21.0661185733841,
-20.2803955927166));
#67956=CARTESIAN_POINT('Ctrl Pts',(-18.5927428468242,-21.0643914004119,
-20.2785901865145));
#67957=CARTESIAN_POINT('Ctrl Pts',(-18.5713020456533,-21.0628482744101,
-20.2773289740498));
#67958=CARTESIAN_POINT('Ctrl Pts',(-18.3711083179642,-21.045371525015,-20.2656286284256));
#67959=CARTESIAN_POINT('Ctrl Pts',(-18.1950414036618,-21.0070974021979,
-20.255986337114));
#67960=CARTESIAN_POINT('Ctrl Pts',(-17.912350610632,-20.9067631532775,-20.2396611387924));
#67961=CARTESIAN_POINT('Ctrl Pts',(-17.8024648994558,-20.8568466047916,
-20.2330507520611));
#67962=CARTESIAN_POINT('Ctrl Pts',(-17.689157601094,-20.7932179504519,-20.2253490632511));
#67963=CARTESIAN_POINT('Ctrl Pts',(-17.6809090873663,-20.7885126467702,
-20.2247830198669));
#67964=CARTESIAN_POINT('Ctrl Pts',(-17.6687291735151,-20.7814556702144,
-20.223938765414));
#67965=CARTESIAN_POINT('Ctrl Pts',(-17.6647731694154,-20.7791463999616,
-20.2236632262537));
#67966=CARTESIAN_POINT('Ctrl Pts',(-17.6577458576165,-20.7750136530059,
-20.2231713438855));
#67967=CARTESIAN_POINT('Ctrl Pts',(-17.6546716392989,-20.77319522501,-20.2229553296198));
#67968=CARTESIAN_POINT('Ctrl Pts',(-17.6480696495257,-20.7692675003106,
-20.2224896238912));
#67969=CARTESIAN_POINT('Ctrl Pts',(-17.6445434662935,-20.7671557382954,
-20.2222397767971));
#67970=CARTESIAN_POINT('Ctrl Pts',(-17.6348213755042,-20.7612948342117,
-20.2215478992606));
#67971=CARTESIAN_POINT('Ctrl Pts',(-17.6286385898594,-20.7575241884657,
-20.2211044970959));
#67972=CARTESIAN_POINT('Ctrl Pts',(-17.594779280346,-20.7366355845876,-20.21865804214));
#67973=CARTESIAN_POINT('Ctrl Pts',(-17.5674825584837,-20.7189139218477,
-20.2166186347703));
#67974=CARTESIAN_POINT('Ctrl Pts',(-17.406223797779,-20.6088554531445,-20.2042125252644));
#67975=CARTESIAN_POINT('Ctrl Pts',(-17.2828649139191,-20.5019569440862,
-20.1932560141197));
#67976=CARTESIAN_POINT('Ctrl Pts',(-17.0940643354825,-20.2958542810069,
-20.1749988331776));
#67977=CARTESIAN_POINT('Ctrl Pts',(-17.0224166834121,-20.2033287611289,
-20.1675581752485));
#67978=CARTESIAN_POINT('Ctrl Pts',(-16.9509757412983,-20.0933665829838,
-20.1595512894083));
#67979=CARTESIAN_POINT('Ctrl Pts',(-16.943312257787,-20.0813053659112,-20.158683316669));
#67980=CARTESIAN_POINT('Ctrl Pts',(-16.9313097914056,-20.061985806313,-20.1573090128665));
#67981=CARTESIAN_POINT('Ctrl Pts',(-16.9268912628633,-20.0547776266239,
-20.1567997537533));
#67982=CARTESIAN_POINT('Ctrl Pts',(-16.9191746526594,-20.0420181868551,
-20.1559043780002));
#67983=CARTESIAN_POINT('Ctrl Pts',(-16.9158585869085,-20.0364779815466,
-20.1555176052367));
#67984=CARTESIAN_POINT('Ctrl Pts',(-16.9090523224986,-20.024987678131,-20.1547195381088));
#67985=CARTESIAN_POINT('Ctrl Pts',(-16.9055657515437,-20.0190355119874,
-20.1543083791258));
#67986=CARTESIAN_POINT('Ctrl Pts',(-16.8966908804898,-20.0037133763836,
-20.1532556708245));
#67987=CARTESIAN_POINT('Ctrl Pts',(-16.8913450922958,-19.9943189168253,
-20.1526156628088));
#67988=CARTESIAN_POINT('Ctrl Pts',(-16.869333938067,-19.9549388419176,-20.149954997782));
#67989=CARTESIAN_POINT('Ctrl Pts',(-16.8533261621608,-19.9245903327816,
-20.1479578695779));
#67990=CARTESIAN_POINT('Ctrl Pts',(-16.8135457967482,-19.8445139893793,
-20.1428137897843));
#67991=CARTESIAN_POINT('Ctrl Pts',(-16.7909643571484,-19.7942224789403,
-20.1397062273577));
#67992=CARTESIAN_POINT('Ctrl Pts',(-16.7295080994084,-19.6416795364478,
-20.1305618125667));
#67993=CARTESIAN_POINT('Ctrl Pts',(-16.6965647880973,-19.5372386551154,
-20.1246736897909));
#67994=CARTESIAN_POINT('Ctrl Pts',(-16.661495369825,-19.3861717633026,-20.1162302648609));
#67995=CARTESIAN_POINT('Ctrl Pts',(-16.6526001440765,-19.3413006095121,
-20.1137296440771));
#67996=CARTESIAN_POINT('Ctrl Pts',(-16.6414616925536,-19.2737007555004,
-20.1099306389502));
#67997=CARTESIAN_POINT('Ctrl Pts',(-16.6381212428452,-19.2511657195745,
-20.1086589341801));
#67998=CARTESIAN_POINT('Ctrl Pts',(-16.635014330211,-19.227588753746,-20.10731904276));
#67999=CARTESIAN_POINT('Ctrl Pts',(-16.6348841801674,-19.226595662919,-20.1072625875172));
#68000=CARTESIAN_POINT('Ctrl Pts',(-16.6324561181456,-19.2079660888138,
-20.1062032014243));
#68001=CARTESIAN_POINT('Ctrl Pts',(-16.6303799032461,-19.1903018723446,
-20.1051931370714));
#68002=CARTESIAN_POINT('Ctrl Pts',(-16.6249807896789,-19.1387743742033,
-20.1022251976505));
#68003=CARTESIAN_POINT('Ctrl Pts',(-16.6222515859022,-19.1048562620928,
-20.1002445439356));
#68004=CARTESIAN_POINT('Ctrl Pts',(-16.6199499410138,-19.0639367655804,
-20.0978069261055));
#68005=CARTESIAN_POINT('Ctrl Pts',(-16.6195931839441,-19.0569824012193,
-20.0973909755966));
#68006=CARTESIAN_POINT('Ctrl Pts',(-16.6190643340273,-19.0455735042,-20.0967056680271));
#68007=CARTESIAN_POINT('Ctrl Pts',(-16.6188719863389,-19.0411199017147,
-20.0964374191126));
#68008=CARTESIAN_POINT('Ctrl Pts',(-16.6185512358395,-19.0331062081705,
-20.0959533717234));
#68009=CARTESIAN_POINT('Ctrl Pts',(-16.6184177515004,-19.0295463752165,
-20.0957378607301));
#68010=CARTESIAN_POINT('Ctrl Pts',(-16.6181464746308,-19.0217889496004,
-20.0952671550356));
#68011=CARTESIAN_POINT('Ctrl Pts',(-16.6180121893519,-19.0175913316322,
-20.0950117718546));
#68012=CARTESIAN_POINT('Ctrl Pts',(-16.6176684706817,-19.0057440228531,
-20.0942891163123));
#68013=CARTESIAN_POINT('Ctrl Pts',(-16.6174880266073,-18.9980936477288,
-20.0938202690771));
#68014=CARTESIAN_POINT('Ctrl Pts',(-16.6166359125984,-18.9511762171222,
-20.0909322144367));
#68015=CARTESIAN_POINT('Ctrl Pts',(-16.6170156060812,-18.9119003966035,
-20.0884598542696));
#68016=CARTESIAN_POINT('Ctrl Pts',(-16.6246864730281,-18.7073629006315,
-20.0753759115104));
#68017=CARTESIAN_POINT('Ctrl Pts',(-16.650236814253,-18.5433629186059,-20.0642279664343));
#68018=CARTESIAN_POINT('Ctrl Pts',(-16.7233108427889,-18.2809906220141,
-20.0465068286882));
#68019=CARTESIAN_POINT('Ctrl Pts',(-16.7597694081222,-18.1802849572855,
-20.0397217322053));
#68020=CARTESIAN_POINT('Ctrl Pts',(-16.809486709708,-18.0698793026648,-20.0323300216615));
#68021=CARTESIAN_POINT('Ctrl Pts',(-16.8154125130484,-18.0570640250555,
-20.0314725683119));
#68022=CARTESIAN_POINT('Ctrl Pts',(-16.8250698839282,-18.0367156432777,
-20.030111726026));
#68023=CARTESIAN_POINT('Ctrl Pts',(-16.8287188044834,-18.0291439923261,
-20.0296054976374));
#68024=CARTESIAN_POINT('Ctrl Pts',(-16.8352469108427,-18.0158016813022,
-20.0287136402764));
#68025=CARTESIAN_POINT('Ctrl Pts',(-16.8381075357463,-18.0100221069842,
-20.028327371423));
#68026=CARTESIAN_POINT('Ctrl Pts',(-16.8440919083803,-17.9980690418548,
-20.0275285986674));
#68027=CARTESIAN_POINT('Ctrl Pts',(-16.8472196044384,-17.991897605279,-20.0271162387682));
#68028=CARTESIAN_POINT('Ctrl Pts',(-16.8553536454317,-17.9760411204043,
-20.0260568146678));
#68029=CARTESIAN_POINT('Ctrl Pts',(-16.8604046918547,-17.9663791356616,
-20.0254113305305));
#68030=CARTESIAN_POINT('Ctrl Pts',(-16.8820452178162,-17.925751221827,-20.0226969196544));
#68031=CARTESIAN_POINT('Ctrl Pts',(-16.8993300412366,-17.8951606446635,
-20.0206527521062));
#68032=CARTESIAN_POINT('Ctrl Pts',(-16.9466054074943,-17.8161515111259,
-20.0153593944998));
#68033=CARTESIAN_POINT('Ctrl Pts',(-16.9778026004702,-17.7684871719808,
-20.0121526604569));
#68034=CARTESIAN_POINT('Ctrl Pts',(-17.0973195531202,-17.6010366452894,
-20.000730128435));
#68035=CARTESIAN_POINT('Ctrl Pts',(-17.1962736690529,-17.4893926877315,
-19.9928376963955));
#68036=CARTESIAN_POINT('Ctrl Pts',(-17.3623928375813,-17.3376288201956,
-19.9803866816486));
#68037=CARTESIAN_POINT('Ctrl Pts',(-17.4214050181273,-17.2892936837539,
-19.9760811738258));
#68038=CARTESIAN_POINT('Ctrl Pts',(-17.4905593141391,-17.2386305962504,
-19.9710006087807));
#68039=CARTESIAN_POINT('Ctrl Pts',(-17.4982690461535,-17.2330618233827,
-19.9704337192039));
#68040=CARTESIAN_POINT('Ctrl Pts',(-17.5097495285106,-17.2248865723154,
-19.96958844097));
#68041=CARTESIAN_POINT('Ctrl Pts',(-17.5134917659741,-17.2222399996534,
-19.9693127336125));
#68042=CARTESIAN_POINT('Ctrl Pts',(-17.5201656867192,-17.2175525317936,
-19.9688206664646));
#68043=CARTESIAN_POINT('Ctrl Pts',(-17.523093969727,-17.2155068829146,-19.9686046365648));
#68044=CARTESIAN_POINT('Ctrl Pts',(-17.529401333355,-17.2111243781189,-19.9681390290221));
#68045=CARTESIAN_POINT('Ctrl Pts',(-17.5327819934348,-17.2087899786362,
-19.9678892964436));
#68046=CARTESIAN_POINT('Ctrl Pts',(-17.542133631928,-17.2023726442709,-19.9671980531526));
#68047=CARTESIAN_POINT('Ctrl Pts',(-17.5481187090696,-17.1983104939588,
-19.9667551747801));
#68048=CARTESIAN_POINT('Ctrl Pts',(-17.5810413238428,-17.1762110857246,
-19.9643168956794));
#68049=CARTESIAN_POINT('Ctrl Pts',(-17.608368080391,-17.1587647973197,-19.9622854205056));
#68050=CARTESIAN_POINT('Ctrl Pts',(-17.7752802366651,-17.05752111551,-19.9498819441189));
#68051=CARTESIAN_POINT('Ctrl Pts',(-17.9237483133758,-16.9894287408592,
-19.9389181278655));
#68052=CARTESIAN_POINT('Ctrl Pts',(-18.1896523479148,-16.902847314526,-19.9206516930896));
#68053=CARTESIAN_POINT('Ctrl Pts',(-18.3035711042056,-16.8759268142901,
-19.9132088157146));
#68054=CARTESIAN_POINT('Ctrl Pts',(-18.4332776908568,-16.8564191044806,
-19.9051998623574));
#68055=CARTESIAN_POINT('Ctrl Pts',(-18.4474299329633,-16.8544369355657,
-19.904331861564));
#68056=CARTESIAN_POINT('Ctrl Pts',(-18.4699857848919,-16.8515103011535,
-19.9029575213937));
#68057=CARTESIAN_POINT('Ctrl Pts',(-18.4783766664683,-16.8504726517761,
-19.9024482537379));
#68058=CARTESIAN_POINT('Ctrl Pts',(-18.4931861919352,-16.8487312584256,
-19.9015528674848));
#68059=CARTESIAN_POINT('Ctrl Pts',(-18.499602218835,-16.8480065658238,-19.9011660927221));
#68060=CARTESIAN_POINT('Ctrl Pts',(-18.5128794096425,-16.8465683893715,
-19.900368025793));
#68061=CARTESIAN_POINT('Ctrl Pts',(-18.5197409539613,-16.8458590632543,
-19.8999568689869));
#68062=CARTESIAN_POINT('Ctrl Pts',(-18.5373623443071,-16.8441244214811,
-19.8989041752007));
#68063=CARTESIAN_POINT('Ctrl Pts',(-18.5481268813494,-16.8431479396425,
-19.8982641794315));
#68064=CARTESIAN_POINT('Ctrl Pts',(-18.5930842496861,-16.8394166379384,
-19.8956036398859));
#68065=CARTESIAN_POINT('Ctrl Pts',(-18.6273351421491,-16.8374105563929,
-19.8936066220194));
#68066=CARTESIAN_POINT('Ctrl Pts',(-18.7166896998723,-16.8343537957907,
-19.8884628926149));
#68067=CARTESIAN_POINT('Ctrl Pts',(-18.7718132900223,-16.8346205127423,
-19.8853555631007));
#68068=CARTESIAN_POINT('Ctrl Pts',(-19.0100756690398,-16.8450824855816,
-19.872094512402));
#68069=CARTESIAN_POINT('Ctrl Pts',(-19.1914406303232,-16.8768962206083,
-19.8625018406128));
#68070=CARTESIAN_POINT('Ctrl Pts',(-19.4105435273638,-16.9454817878797,
-19.8495094779168));
#68071=CARTESIAN_POINT('Ctrl Pts',(-19.4541974694506,-16.9607337207652,
-19.8468428909266));
#68072=CARTESIAN_POINT('Ctrl Pts',(-19.5044480534193,-16.980158904741,-19.8436436569624));
#68073=CARTESIAN_POINT('Ctrl Pts',(-19.5115674651876,-16.9829554750961,
-19.843187308468));
#68074=CARTESIAN_POINT('Ctrl Pts',(-19.5229582137532,-16.9875012751231,
-19.8424519725694));
#68075=CARTESIAN_POINT('Ctrl Pts',(-19.5272393316553,-16.9892260280709,
-19.842174419653));
#68076=CARTESIAN_POINT('Ctrl Pts',(-19.5348348349426,-16.992314970882,-19.8416798264017));
#68077=CARTESIAN_POINT('Ctrl Pts',(-19.5381514343886,-16.9936735929365,
-19.8414631240229));
#68078=CARTESIAN_POINT('Ctrl Pts',(-19.5451998894675,-16.9965818690275,
-19.8410009980104));
#68079=CARTESIAN_POINT('Ctrl Pts',(-19.5489307051641,-16.9981337628289,
-19.8407554449695));
#68080=CARTESIAN_POINT('Ctrl Pts',(-19.558917228362,-17.0023213988837,-19.8400956656079));
#68081=CARTESIAN_POINT('Ctrl Pts',(-19.5651646779393,-17.0049765392887,
-19.8396802888679));
#68082=CARTESIAN_POINT('Ctrl Pts',(-19.5960844743466,-17.0182932601736,
-19.8376118515134));
#68083=CARTESIAN_POINT('Ctrl Pts',(-19.6205637811342,-17.0293934615107,
-19.8359341776948));
#68084=CARTESIAN_POINT('Ctrl Pts',(-19.6907536179436,-17.0628466800175,
-19.8310206464795));
#68085=CARTESIAN_POINT('Ctrl Pts',(-19.7358764250408,-17.086384635568,-19.82773328606));
#68086=CARTESIAN_POINT('Ctrl Pts',(-19.8667078395912,-17.1607476024165,
-19.8179014967938));
#68087=CARTESIAN_POINT('Ctrl Pts',(-19.9497283289733,-17.2160227873667,
-19.8112717116829));
#68088=CARTESIAN_POINT('Ctrl Pts',(-20.0405380766754,-17.2862038346826,
-19.803731910975));
#68089=CARTESIAN_POINT('Ctrl Pts',(-20.0524279870393,-17.2955983994748,
-19.802738437101));
#68090=CARTESIAN_POINT('Ctrl Pts',(-20.1576039360046,-17.3805509977562,
-19.7938970945792));
#68091=CARTESIAN_POINT('Ctrl Pts',(-20.2444184714402,-17.4637981947573,
-19.7862404440536));
#68092=CARTESIAN_POINT('Ctrl Pts',(-20.334095497553,-17.5657711831682,-19.7779483908196));
#68093=CARTESIAN_POINT('Ctrl Pts',(-20.3443413328403,-17.5776868091483,
-19.7769943256731));
#68094=CARTESIAN_POINT('Ctrl Pts',(-20.3596415887045,-17.5958866494414,
-19.7755590871145));
#68095=CARTESIAN_POINT('Ctrl Pts',(-20.3647941742819,-17.6020872774793,
-19.7750738944653));
#68096=CARTESIAN_POINT('Ctrl Pts',(-20.3739636688635,-17.6132509837842,
-19.7742070446102));
#68097=CARTESIAN_POINT('Ctrl Pts',(-20.377993761708,-17.6182030602599,-19.7738248544275));
#68098=CARTESIAN_POINT('Ctrl Pts',(-20.3864973809088,-17.6287491886064,
-19.7730158217329));
#68099=CARTESIAN_POINT('Ctrl Pts',(-20.3909650520357,-17.6343478751839,
-19.772589217814));
#68100=CARTESIAN_POINT('Ctrl Pts',(-20.4028443464048,-17.6493904413009,
-19.771450648905));
#68101=CARTESIAN_POINT('Ctrl Pts',(-20.4102042683554,-17.6588749578475,
-19.770740747503));
#68102=CARTESIAN_POINT('Ctrl Pts',(-20.4456332339009,-17.7053419868914,
-19.76730060182));
#68103=CARTESIAN_POINT('Ctrl Pts',(-20.4725624463873,-17.743180071677,-19.7646151981559));
#68104=CARTESIAN_POINT('Ctrl Pts',(-20.5482263636716,-17.857260510455,-19.7568168015629));
#68105=CARTESIAN_POINT('Ctrl Pts',(-20.5933452475915,-17.9357770445965,
-19.7518286380275));
#68106=CARTESIAN_POINT('Ctrl Pts',(-20.6664468123528,-18.0842624367219,
-19.7428027245657));
#68107=CARTESIAN_POINT('Ctrl Pts',(-20.6959858739097,-18.1532945405059,
-19.7387530398212));
#68108=CARTESIAN_POINT('Ctrl Pts',(-20.7571087062752,-18.3201322190897,
-19.7290386426034));
#68109=CARTESIAN_POINT('Ctrl Pts',(-20.785358515489,-18.4189443609152,-19.7233418224833));
#68110=CARTESIAN_POINT('Ctrl Pts',(-20.8083088064251,-18.5288855092317,
-19.716687994081));
#68111=CARTESIAN_POINT('Ctrl Pts',(-20.8102237312023,-18.5383843491317,
-19.7161105530016));
#68112=CARTESIAN_POINT('Ctrl Pts',(-20.8129549517807,-18.5524294310593,
-19.7152525289895));
#68113=CARTESIAN_POINT('Ctrl Pts',(-20.8138217188903,-18.5569658903304,
-19.7149747460142));
#68114=CARTESIAN_POINT('Ctrl Pts',(-20.8153331726451,-18.5650193680193,
-19.7144803978423));
#68115=CARTESIAN_POINT('Ctrl Pts',(-20.8159838012209,-18.5685352215321,
-19.7142641742975));
#68116=CARTESIAN_POINT('Ctrl Pts',(-20.8173588170755,-18.5760721708738,
-19.7137997612742));
#68117=CARTESIAN_POINT('Ctrl Pts',(-20.8180804607375,-18.5800936597507,
-19.7135514253113));
#68118=CARTESIAN_POINT('Ctrl Pts',(-20.819537503568,-18.5883507154137,-19.7130404633478));
#68119=CARTESIAN_POINT('Ctrl Pts',(-20.8202716512641,-18.5925864813869,
-19.7127777691835));
#68120=CARTESIAN_POINT('Ctrl Pts',(-20.8220969243962,-18.6033116893226,
-19.7121112034224));
#68121=CARTESIAN_POINT('Ctrl Pts',(-20.8231706938927,-18.6098039846676,
-19.7117064072045));
#68122=CARTESIAN_POINT('Ctrl Pts',(-20.8419516469325,-18.7267427419427,
-19.704393091252));
#68123=CARTESIAN_POINT('Ctrl Pts',(-20.8509055118865,-18.8384008838167,
-19.6970632585576));
#68124=CARTESIAN_POINT('Ctrl Pts',(-20.8509992561137,-18.9502252848438,
-19.6896814721675));
#68125=CARTESIAN_POINT('Ctrl Pts',(-20.8509992546728,-18.9502235668445,
-19.6896815855766));
#68126=CARTESIAN_POINT('Ctrl Pts',(-20.8510836457028,-19.0507934909693,
-19.6830427336087));
#68127=CARTESIAN_POINT('Ctrl Pts',(-20.844001378845,-19.1512504950245,-19.6763789318511));
#68128=CARTESIAN_POINT('Ctrl Pts',(-20.8172660724819,-19.3387551736086,
-19.6641118465099));
#68129=CARTESIAN_POINT('Ctrl Pts',(-20.7992074267082,-19.4258130985577,
-19.658486560603));
#68130=CARTESIAN_POINT('Ctrl Pts',(-20.7702875631048,-19.5313496542403,
-19.6517704142229));
#68131=CARTESIAN_POINT('Ctrl Pts',(-20.7645555899519,-19.5511302902294,
-19.6505158868579));
#68132=CARTESIAN_POINT('Ctrl Pts',(-20.755942028075,-19.5793102638725,-19.6487342543039));
#68133=CARTESIAN_POINT('Ctrl Pts',(-20.7532949575033,-19.5877795297144,
-19.648199525735));
#68134=CARTESIAN_POINT('Ctrl Pts',(-20.7486160613219,-19.6024255533593,
-19.6472760010289));
#68135=CARTESIAN_POINT('Ctrl Pts',(-20.7466088978239,-19.6086100066726,
-19.646886401071));
#68136=CARTESIAN_POINT('Ctrl Pts',(-20.7426965192785,-19.6204782922701,
-19.6461394126603));
#68137=CARTESIAN_POINT('Ctrl Pts',(-20.7407955948982,-19.6261634632885,
-19.6457818872301));
#68138=CARTESIAN_POINT('Ctrl Pts',(-20.7357563731666,-19.6410242824532,
-19.644848069307));
#68139=CARTESIAN_POINT('Ctrl Pts',(-20.7325791090231,-19.6501866434224,
-19.6442730699062));
#68140=CARTESIAN_POINT('Ctrl Pts',(-20.727115684882,-19.6655987280105,-19.6433069814357));
#68141=CARTESIAN_POINT('Ctrl Pts',(-20.7248628673184,-19.671859931052,-19.6429148193411));
#68142=CARTESIAN_POINT('Ctrl Pts',(-20.7225805821918,-19.6781103691105,
-19.6425236185391));
#68143=CARTESIAN_POINT('Origin',(-18.734,-18.952,0.));
#68144=CARTESIAN_POINT('',(-20.7225806288389,-19.6781102413592,-18.845275429269));
#68145=CARTESIAN_POINT('',(-20.7225805821191,-19.6781103693095,-19.0663245248053));
#68146=CARTESIAN_POINT('',(-20.7225805821191,-19.6781103693095,0.));
#68147=CARTESIAN_POINT('',(-20.8499619975019,-18.9538841873159,-19.1109437209775));
#68148=CARTESIAN_POINT('Ctrl Pts',(-20.7225805821191,-19.6781103693095,
-19.0663245248053));
#68149=CARTESIAN_POINT('Ctrl Pts',(-20.7389260930203,-19.6333453212442,
-19.0692018319792));
#68150=CARTESIAN_POINT('Ctrl Pts',(-20.7537412767065,-19.5880774322525,
-19.0720791391531));
#68151=CARTESIAN_POINT('Ctrl Pts',(-20.7670007520339,-19.5424209872875,
-19.074956446327));
#68152=CARTESIAN_POINT('Ctrl Pts',(-20.7921933233411,-19.4556752287257,
-19.0804232362535));
#68153=CARTESIAN_POINT('Ctrl Pts',(-20.8118478930247,-19.3672535084955,
-19.0858900261801));
#68154=CARTESIAN_POINT('Ctrl Pts',(-20.8257819138129,-19.2777873923974,
-19.0913568161066));
#68155=CARTESIAN_POINT('Ctrl Pts',(-20.839488073104,-19.1897843057774,-19.0967342082235));
#68156=CARTESIAN_POINT('Ctrl Pts',(-20.8476592207516,-19.1007706087727,
-19.1021116003405));
#68157=CARTESIAN_POINT('Ctrl Pts',(-20.8501673751619,-19.0113686811404,
-19.1074889924574));
#68158=CARTESIAN_POINT('Ctrl Pts',(-20.8507044999978,-18.9922231311271,
-19.1086405686307));
#68159=CARTESIAN_POINT('Ctrl Pts',(-20.8509820862726,-18.9730598582293,
-19.1097921448041));
#68160=CARTESIAN_POINT('Ctrl Pts',(-20.8509991606888,-18.9538851108721,
-19.1109437209775));
#68161=CARTESIAN_POINT('Ctrl Pts',(-20.8499619975019,-18.9538841873159,
-19.1109437209775));
#68162=CARTESIAN_POINT('Ctrl Pts',(-20.8456331448199,-18.4480050364302,
-19.1413398983212));
#68163=CARTESIAN_POINT('Ctrl Pts',(-20.4101935050426,-17.2299119675837,
-19.2141280112252));
#68164=CARTESIAN_POINT('Ctrl Pts',(-18.3741968410994,-16.4747290082863,
-19.3293080596899));
#68165=CARTESIAN_POINT('Ctrl Pts',(-16.456252502104,-17.9136376975396,-19.4564838663714));
#68166=CARTESIAN_POINT('Ctrl Pts',(-16.6280001175491,-20.3051793956671,
-19.5836596730528));
#68167=CARTESIAN_POINT('Ctrl Pts',(-18.7318719157577,-21.4552629005109,
-19.7108354797342));
#68168=CARTESIAN_POINT('Ctrl Pts',(-20.2929104233135,-20.6053638626281,
-19.8051103644544));
#68169=CARTESIAN_POINT('Ctrl Pts',(-20.6701804022281,-19.8268832656859,
-19.8569933136142));
#68170=CARTESIAN_POINT('Ctrl Pts',(-20.7227693935251,-19.6781792853784,
-19.8664843272136));
#68171=CARTESIAN_POINT('Ctrl Pts',(-20.7225805821918,-19.6781103691105,
-19.6425236185391));
#68172=CARTESIAN_POINT('Ctrl Pts',(-20.7166653576808,-19.6943102487738,
-19.641509704657));
#68173=CARTESIAN_POINT('Ctrl Pts',(-20.710552187151,-19.7104378159453,-19.6405022550434));
#68174=CARTESIAN_POINT('Ctrl Pts',(-20.6468793838964,-19.8724165912212,
-19.630397967332));
#68175=CARTESIAN_POINT('Ctrl Pts',(-20.5734821739296,-20.0115218277049,
-19.6218861304148));
#68176=CARTESIAN_POINT('Ctrl Pts',(-20.4399820734497,-20.2081237322731,
-19.6089797865278));
#68177=CARTESIAN_POINT('Ctrl Pts',(-20.3907876123171,-20.2723314550053,
-19.6045896005813));
#68178=CARTESIAN_POINT('Ctrl Pts',(-20.3116702093477,-20.3641895034725,
-19.597801964565));
#68179=CARTESIAN_POINT('Ctrl Pts',(-20.2844242310254,-20.3940495134181,
-19.5955064655122));
#68180=CARTESIAN_POINT('Ctrl Pts',(-20.2404516176395,-20.4395535058783,
-19.5918318001489));
#68181=CARTESIAN_POINT('Ctrl Pts',(-20.2242964647885,-20.4557380955299,
-19.5904877078463));
#68182=CARTESIAN_POINT('Ctrl Pts',(-20.2032487008755,-20.476151874231,-19.5887389696148));
#68183=CARTESIAN_POINT('Ctrl Pts',(-20.1985938433898,-20.4806253799376,
-19.5883523717303));
#68184=CARTESIAN_POINT('Ctrl Pts',(-20.1914747000028,-20.4874047962422,
-19.5877611959693));
#68185=CARTESIAN_POINT('Ctrl Pts',(-20.1890251926361,-20.4897262688464,
-19.5875578037743));
#68186=CARTESIAN_POINT('Ctrl Pts',(-20.1839774699174,-20.4944872897189,
-19.587138677327));
#68187=CARTESIAN_POINT('Ctrl Pts',(-20.1813786655035,-20.4969261148266,
-19.5869228906763));
#68188=CARTESIAN_POINT('Ctrl Pts',(-20.1754965377455,-20.5024182773035,
-19.5864344824733));
#68189=CARTESIAN_POINT('Ctrl Pts',(-20.1722096841926,-20.5054677358632,
-19.5861615726575));
#68190=CARTESIAN_POINT('Ctrl Pts',(-20.1625003659489,-20.514418567213,-19.5853554863338));
#68191=CARTESIAN_POINT('Ctrl Pts',(-20.1560511801885,-20.5202906330141,
-19.5848201719844));
#68192=CARTESIAN_POINT('Ctrl Pts',(-20.1098730376359,-20.5618173928256,
-19.5809891224532));
#68193=CARTESIAN_POINT('Ctrl Pts',(-20.0688475906991,-20.5959949895138,
-19.5775961909825));
#68194=CARTESIAN_POINT('Ctrl Pts',(-20.0127922062523,-20.6392114662941,
-19.5730216044894));
#68195=CARTESIAN_POINT('Ctrl Pts',(-19.9988754170776,-20.6496696364701,
-19.5718906194675));
#68196=CARTESIAN_POINT('Ctrl Pts',(-19.8572280126433,-20.7534060115647,
-19.5604380159078));
#68197=CARTESIAN_POINT('Ctrl Pts',(-19.7195362708858,-20.8322741708811,
-19.549832160147));
#68198=CARTESIAN_POINT('Ctrl Pts',(-19.5237780860885,-20.9169363262836,
-19.5361230744716));
#68199=CARTESIAN_POINT('Ctrl Pts',(-19.4723744528574,-20.9368244707487,
-19.5326344323805));
#68200=CARTESIAN_POINT('Ctrl Pts',(-19.3878021241933,-20.965804423035,-19.5270775586395));
#68201=CARTESIAN_POINT('Ctrl Pts',(-19.3550877111118,-20.9761333313784,
-19.5249709002405));
#68202=CARTESIAN_POINT('Ctrl Pts',(-19.3117525959949,-20.9886658419112,
-19.522234597395));
#68203=CARTESIAN_POINT('Ctrl Pts',(-19.3013470283985,-20.9915889708319,
-19.5215816164418));
#68204=CARTESIAN_POINT('Ctrl Pts',(-19.2842644208192,-20.9962469636859,
-19.5205161453214));
#68205=CARTESIAN_POINT('Ctrl Pts',(-19.2776005744641,-20.9980290805736,
-19.520102125869));
#68206=CARTESIAN_POINT('Ctrl Pts',(-19.2646824261088,-21.0014162223706,
-19.5193026139653));
#68207=CARTESIAN_POINT('Ctrl Pts',(-19.2584292655106,-21.0030252647879,
-19.5189169952063));
#68208=CARTESIAN_POINT('Ctrl Pts',(-19.2439711248367,-21.0066751412676,
-19.5180285609203));
#68209=CARTESIAN_POINT('Ctrl Pts',(-19.2357610495381,-21.0086954895269,
-19.5175264115259));
#68210=CARTESIAN_POINT('Ctrl Pts',(-19.213642289766,-21.0139981793584,-19.516179748457));
#68211=CARTESIAN_POINT('Ctrl Pts',(-19.1997119578373,-21.0171889998374,
-19.5153381765576));
#68212=CARTESIAN_POINT('Ctrl Pts',(-19.0715533720643,-21.0451817361065,
-19.507653217771));
#68213=CARTESIAN_POINT('Ctrl Pts',(-18.9554801047576,-21.0606260671115,
-19.5011268231189));
#68214=CARTESIAN_POINT('Ctrl Pts',(-18.6759634182878,-21.0744685344132,
-19.4858063384499));
#68215=CARTESIAN_POINT('Ctrl Pts',(-18.5128492471517,-21.0637105212473,
-19.4771959195974));
#68216=CARTESIAN_POINT('Ctrl Pts',(-18.3208634474756,-21.0285472405061,
-19.4659860531521));
#68217=CARTESIAN_POINT('Ctrl Pts',(-18.2892619825469,-21.0220092011954,
-19.4641036529904));
#68218=CARTESIAN_POINT('Ctrl Pts',(-18.2507862158518,-21.0131272674601,
-19.4617524356487));
#68219=CARTESIAN_POINT('Ctrl Pts',(-18.2437566378528,-21.0114665853829,
-19.4613204217365));
#68220=CARTESIAN_POINT('Ctrl Pts',(-18.2327446160162,-21.0088055085237,
-19.4606396275385));
#68221=CARTESIAN_POINT('Ctrl Pts',(-18.2287562736889,-21.0078294278054,
-19.4603922250205));
#68222=CARTESIAN_POINT('Ctrl Pts',(-18.2213032589949,-21.0059824279431,
-19.4599283040653));
#68223=CARTESIAN_POINT('Ctrl Pts',(-18.2178379428988,-21.0051143398958,
-19.45971194965));
#68224=CARTESIAN_POINT('Ctrl Pts',(-18.2099281801634,-21.0031115933003,
-19.4592166284064));
#68225=CARTESIAN_POINT('Ctrl Pts',(-18.205485228663,-21.0019712622575,-19.4589373378272));
#68226=CARTESIAN_POINT('Ctrl Pts',(-18.1938960459762,-20.9989565947872,
-19.4582061026457));
#68227=CARTESIAN_POINT('Ctrl Pts',(-18.1867559296653,-20.9970592915401,
-19.45775288038));
#68228=CARTESIAN_POINT('Ctrl Pts',(-18.1399886753272,-20.9843696355961,
-19.4547671946653));
#68229=CARTESIAN_POINT('Ctrl Pts',(-18.1006756117236,-20.9724641787672,
-19.452176767735));
#68230=CARTESIAN_POINT('Ctrl Pts',(-18.0519404954401,-20.9561433487171,
-19.4488846754571));
#68231=CARTESIAN_POINT('Ctrl Pts',(-18.0421684963805,-20.9527910671409,
-19.4482204356643));
#68232=CARTESIAN_POINT('Ctrl Pts',(-18.0097868094912,-20.9414169491303,
-19.4460063895182));
#68233=CARTESIAN_POINT('Ctrl Pts',(-17.9872894114241,-20.9330824765389,
-19.4444471234952));
#68234=CARTESIAN_POINT('Ctrl Pts',(-17.837498545487,-20.8746763831487,-19.4339432249352));
#68235=CARTESIAN_POINT('Ctrl Pts',(-17.7151635432548,-20.812745882073,-19.4247959430838));
#68236=CARTESIAN_POINT('Ctrl Pts',(-17.515232337629,-20.6858665341907,-19.4094446777633));
#68237=CARTESIAN_POINT('Ctrl Pts',(-17.43469764991,-20.6263674018111,-19.4031231743271));
#68238=CARTESIAN_POINT('Ctrl Pts',(-17.3474673331981,-20.5518227933746,
-19.3961265280556));
#68239=CARTESIAN_POINT('Ctrl Pts',(-17.3363734622376,-20.5421402090508,
-19.3952335088317));
#68240=CARTESIAN_POINT('Ctrl Pts',(-17.3195949635958,-20.5271849018764,
-19.3938777331764));
#68241=CARTESIAN_POINT('Ctrl Pts',(-17.3138369481387,-20.5219955384412,
-19.3934115136352));
#68242=CARTESIAN_POINT('Ctrl Pts',(-17.3034061506601,-20.5124905300312,
-19.3925651587053));
#68243=CARTESIAN_POINT('Ctrl Pts',(-17.2987240895855,-20.5081852455403,
-19.3921845923967));
#68244=CARTESIAN_POINT('Ctrl Pts',(-17.2886503339771,-20.4988380110578,
-19.3913642997511));
#68245=CARTESIAN_POINT('Ctrl Pts',(-17.2832654510902,-20.4937888183022,
-19.3909248896101));
#68246=CARTESIAN_POINT('Ctrl Pts',(-17.2687174369311,-20.480004018176,-19.3897351486828));
#68247=CARTESIAN_POINT('Ctrl Pts',(-17.2596059848029,-20.4712141282978,
-19.3889871683275));
#68248=CARTESIAN_POINT('Ctrl Pts',(-17.2154438680406,-20.4278390493299,
-19.3853468848612));
#68249=CARTESIAN_POINT('Ctrl Pts',(-17.1815266991841,-20.3921183385539,
-19.382505046357));
#68250=CARTESIAN_POINT('Ctrl Pts',(-17.1219087889954,-20.3247735098996,
-19.3773957271431));
#68251=CARTESIAN_POINT('Ctrl Pts',(-17.0958168402788,-20.2935294852072,
-19.3751151727469));
#68252=CARTESIAN_POINT('Ctrl Pts',(-16.9975791072514,-20.1687504010045,
-19.3663044334865));
#68253=CARTESIAN_POINT('Ctrl Pts',(-16.9324124845035,-20.0699990351479,
-19.3599702655939));
#68254=CARTESIAN_POINT('Ctrl Pts',(-16.8401700281487,-19.9010170997785,
-19.3494529209928));
#68255=CARTESIAN_POINT('Ctrl Pts',(-16.8079896850523,-19.8338775324443,
-19.3453447514761));
#68256=CARTESIAN_POINT('Ctrl Pts',(-16.7661824035679,-19.7333892696328,
-19.3391085907452));
#68257=CARTESIAN_POINT('Ctrl Pts',(-16.7537311183882,-19.701273069552,-19.3371027601424));
#68258=CARTESIAN_POINT('Ctrl Pts',(-16.7395747353296,-19.6619374218935,
-19.3346143329801));
#68259=CARTESIAN_POINT('Ctrl Pts',(-16.7371161760444,-19.6549923679253,
-19.334173793948));
#68260=CARTESIAN_POINT('Ctrl Pts',(-16.7333335382878,-19.6441270330578,
-19.333482528196));
#68261=CARTESIAN_POINT('Ctrl Pts',(-16.7319845897272,-19.6402153858105,
-19.3332332500647));
#68262=CARTESIAN_POINT('Ctrl Pts',(-16.7294937195895,-19.6329231266423,
-19.3327677203345));
#68263=CARTESIAN_POINT('Ctrl Pts',(-16.72834887434,-19.6295435735896,-19.3325516444486));
#68264=CARTESIAN_POINT('Ctrl Pts',(-16.7257666516426,-19.6218570255782,
-19.3320594556358));
#68265=CARTESIAN_POINT('Ctrl Pts',(-16.724334589348,-19.6175483096756,-19.3317830348896));
#68266=CARTESIAN_POINT('Ctrl Pts',(-16.7201090336721,-19.6046966838548,
-19.3309570680216));
#68267=CARTESIAN_POINT('Ctrl Pts',(-16.7173561142753,-19.596140681044,-19.3304052269574));
#68268=CARTESIAN_POINT('Ctrl Pts',(-16.6964356281362,-19.5296715576422,
-19.3261044521384));
#68269=CARTESIAN_POINT('Ctrl Pts',(-16.6807134772718,-19.4710240846937,
-19.3222300748775));
#68270=CARTESIAN_POINT('Ctrl Pts',(-16.6545294519615,-19.3533430424406,
-19.3144035907617));
#68271=CARTESIAN_POINT('Ctrl Pts',(-16.6440111142916,-19.2943740081285,
-19.3104566838939));
#68272=CARTESIAN_POINT('Ctrl Pts',(-16.6214535394725,-19.1271696831847,
-19.2993103664967));
#68273=CARTESIAN_POINT('Ctrl Pts',(-16.6152406948084,-19.0183283631444,
-19.2921162118095));
#68274=CARTESIAN_POINT('Ctrl Pts',(-16.6189300604191,-18.8346522259922,
-19.2803137415875));
#68275=CARTESIAN_POINT('Ctrl Pts',(-16.6244009300767,-18.7599446834037,
-19.2756050152667));
#68276=CARTESIAN_POINT('Ctrl Pts',(-16.6361817721213,-18.6670430439444,
-19.2698683995353));
#68277=CARTESIAN_POINT('Ctrl Pts',(-16.6387925924027,-18.6484415396243,
-19.2687256112206));
#68278=CARTESIAN_POINT('Ctrl Pts',(-16.6429516208518,-18.6214265985706,
-19.2670740193754));
#68279=CARTESIAN_POINT('Ctrl Pts',(-16.6443037408855,-18.6129842987943,
-19.2665590394248));
#68280=CARTESIAN_POINT('Ctrl Pts',(-16.6467653338031,-18.5981892719056,
-19.2656584967923));
#68281=CARTESIAN_POINT('Ctrl Pts',(-16.647852751649,-18.5918330349496,-19.2652722397606));
#68282=CARTESIAN_POINT('Ctrl Pts',(-16.6500216555879,-18.5794946800263,
-19.2645236566506));
#68283=CARTESIAN_POINT('Ctrl Pts',(-16.6510998977407,-18.5735120628327,
-19.2641612316269));
#68284=CARTESIAN_POINT('Ctrl Pts',(-16.6537407757032,-18.5592123036426,
-19.2632962269793));
#68285=CARTESIAN_POINT('Ctrl Pts',(-16.6553275502313,-18.5508996828545,
-19.2627944194819));
#68286=CARTESIAN_POINT('Ctrl Pts',(-16.6612438231142,-18.5208845092304,
-19.2609860382192));
#68287=CARTESIAN_POINT('Ctrl Pts',(-16.6658638016498,-18.4992401798635,
-19.2596887196481));
#68288=CARTESIAN_POINT('Ctrl Pts',(-16.7123557174045,-18.2970151243205,
-19.2476207470718));
#68289=CARTESIAN_POINT('Ctrl Pts',(-16.7774332190802,-18.1226006641512,
-19.2377043115437));
#68290=CARTESIAN_POINT('Ctrl Pts',(-16.9020631158015,-17.887978516093,-19.2232222275414));
#68291=CARTESIAN_POINT('Ctrl Pts',(-16.9437254532753,-17.8192822510152,
-19.2188075830982));
#68292=CARTESIAN_POINT('Ctrl Pts',(-17.0096095335596,-17.7233961414507,
-19.2121531256959));
#68293=CARTESIAN_POINT('Ctrl Pts',(-17.0307903660063,-17.694197744066,-19.2100552283183));
#68294=CARTESIAN_POINT('Ctrl Pts',(-17.0572435838098,-17.6596251704274,
-19.2074646073566));
#68295=CARTESIAN_POINT('Ctrl Pts',(-17.0618133029625,-17.6537178943589,
-19.2070180967292));
#68296=CARTESIAN_POINT('Ctrl Pts',(-17.0689767432219,-17.6445582771865,
-19.2063195004738));
#68297=CARTESIAN_POINT('Ctrl Pts',(-17.0715490068382,-17.6412891246286,
-19.2060689139591));
#68298=CARTESIAN_POINT('Ctrl Pts',(-17.07634410704,-17.6352317379793,-19.2056022310631));
#68299=CARTESIAN_POINT('Ctrl Pts',(-17.0785643589448,-17.632441531023,-19.2053863184497));
#68300=CARTESIAN_POINT('Ctrl Pts',(-17.0836086488511,-17.6261351023063,
-19.2048961737008));
#68301=CARTESIAN_POINT('Ctrl Pts',(-17.0864368654595,-17.622622305093,-19.20462164427));
#68302=CARTESIAN_POINT('Ctrl Pts',(-17.0937677154814,-17.6135763215634,
-19.2039108419476));
#68303=CARTESIAN_POINT('Ctrl Pts',(-17.0982870892332,-17.6080568611652,
-19.2034734031579));
#68304=CARTESIAN_POINT('Ctrl Pts',(-17.1262011774338,-17.5743150713616,
-19.2007767533001));
#68305=CARTESIAN_POINT('Ctrl Pts',(-17.150296290211,-17.5466833087354,-19.1984713749365));
#68306=CARTESIAN_POINT('Ctrl Pts',(-17.2905170531057,-17.3940687675811,
-19.1852451970303));
#68307=CARTESIAN_POINT('Ctrl Pts',(-17.4206992528575,-17.282857403795,-19.1737337219581));
#68308=CARTESIAN_POINT('Ctrl Pts',(-17.6422278129316,-17.1357376190495,
-19.1564523379592));
#68309=CARTESIAN_POINT('Ctrl Pts',(-17.7251142125269,-17.0884203111888,
-19.1503961515445));
#68310=CARTESIAN_POINT('Ctrl Pts',(-17.8301630321998,-17.0375222586462,
-19.1432260059483));
#68311=CARTESIAN_POINT('Ctrl Pts',(-17.8495480862174,-17.0284898878957,
-19.1419225599029));
#68312=CARTESIAN_POINT('Ctrl Pts',(-17.8772896192678,-17.0160719337491,
-19.1400844149171));
#68313=CARTESIAN_POINT('Ctrl Pts',(-17.8855355006895,-17.0124438261594,
-19.1395414139044));
#68314=CARTESIAN_POINT('Ctrl Pts',(-17.8997945231754,-17.0062783311374,
-19.1386081574022));
#68315=CARTESIAN_POINT('Ctrl Pts',(-17.9057966516453,-17.0037159330579,
-19.1382170514343));
#68316=CARTESIAN_POINT('Ctrl Pts',(-17.9173073022399,-16.9988646697857,
-19.1374702809543));
#68317=CARTESIAN_POINT('Ctrl Pts',(-17.9228138280109,-16.996571255146,-19.1371144646156));
#68318=CARTESIAN_POINT('Ctrl Pts',(-17.937148406578,-16.9906720130187,-19.1361918660068));
#68319=CARTESIAN_POINT('Ctrl Pts',(-17.9459913232665,-16.9871024799316,
-19.1356263158361));
#68320=CARTESIAN_POINT('Ctrl Pts',(-17.9761779552821,-16.9751539016862,
-19.1337076838583));
#68321=CARTESIAN_POINT('Ctrl Pts',(-17.997634016078,-16.9670617273971,-19.1323642327048));
#68322=CARTESIAN_POINT('Ctrl Pts',(-18.1851717970417,-16.8997912144435,
-19.1207861084486));
#68323=CARTESIAN_POINT('Ctrl Pts',(-18.357909126627,-16.8612260736904,-19.111310598646));
#68324=CARTESIAN_POINT('Ctrl Pts',(-18.6194791893889,-16.8363338261108,
-19.0970121190958));
#68325=CARTESIAN_POINT('Ctrl Pts',(-18.7059301568894,-16.8334230960824,
-19.0922789500323));
#68326=CARTESIAN_POINT('Ctrl Pts',(-18.8299712795888,-16.83684090002,-19.0851931276914));
#68327=CARTESIAN_POINT('Ctrl Pts',(-18.8675963009726,-16.838883784974,-19.0830043730105));
#68328=CARTESIAN_POINT('Ctrl Pts',(-18.9126826185291,-16.8425406556746,
-19.0803129997573));
#68329=CARTESIAN_POINT('Ctrl Pts',(-18.9202177044491,-16.8431924776871,
-19.0798608942191));
#68330=CARTESIAN_POINT('Ctrl Pts',(-18.9319119053231,-16.8442672480035,
-19.0791554335674));
#68331=CARTESIAN_POINT('Ctrl Pts',(-18.9360736205007,-16.8446621705784,
-19.078903625593));
#68332=CARTESIAN_POINT('Ctrl Pts',(-18.9437810865531,-16.8454166056384,
-19.0784358449493));
#68333=CARTESIAN_POINT('Ctrl Pts',(-18.9473271095425,-16.8457727460157,
-19.0782200635003));
#68334=CARTESIAN_POINT('Ctrl Pts',(-18.955331123892,-16.8465970394489,-19.0777317305294));
#68335=CARTESIAN_POINT('Ctrl Pts',(-18.9597885121036,-16.8470703955601,
-19.077458891137));
#68336=CARTESIAN_POINT('Ctrl Pts',(-18.9729093915315,-16.8485059341782,
-19.0766532012215));
#68337=CARTESIAN_POINT('Ctrl Pts',(-18.9815683593811,-16.8495074592901,
-19.0761182159341));
#68338=CARTESIAN_POINT('Ctrl Pts',(-19.0431255462348,-16.8570129055434,
-19.0722928079547));
#68339=CARTESIAN_POINT('Ctrl Pts',(-19.0957633011967,-16.8654584093374,
-19.0689054950545));
#68340=CARTESIAN_POINT('Ctrl Pts',(-19.1656388383923,-16.8793930337781,
-19.0643007329114));
#68341=CARTESIAN_POINT('Ctrl Pts',(-19.1832106628471,-16.8831303864347,
-19.0631334583941));
#68342=CARTESIAN_POINT('Ctrl Pts',(-19.247762684622,-16.8977211115999,-19.0588155672159));
#68343=CARTESIAN_POINT('Ctrl Pts',(-19.2944148912027,-16.9099547594957,
-19.0556369323652));
#68344=CARTESIAN_POINT('Ctrl Pts',(-19.4454004603957,-16.9551118536413,
-19.0452267183417));
#68345=CARTESIAN_POINT('Ctrl Pts',(-19.5476150532436,-16.9945304867991,
-19.0379941552358));
#68346=CARTESIAN_POINT('Ctrl Pts',(-19.7146197639511,-17.0742883792042,
-19.0260981926706));
#68347=CARTESIAN_POINT('Ctrl Pts',(-19.7811167750216,-17.1105427750303,
-19.02133540524));
#68348=CARTESIAN_POINT('Ctrl Pts',(-19.8616163712297,-17.1602055579949,
-19.0155404663254));
#68349=CARTESIAN_POINT('Ctrl Pts',(-19.8775637900329,-17.1703412511018,
-19.0143907715948));
#68350=CARTESIAN_POINT('Ctrl Pts',(-19.9005446215904,-17.1853828666926,
-19.012731102403));
#68351=CARTESIAN_POINT('Ctrl Pts',(-19.9076869637124,-17.1901199347167,
-19.0122148662593));
#68352=CARTESIAN_POINT('Ctrl Pts',(-19.9201552883205,-17.1984988576672,
-19.0113128741283));
#68353=CARTESIAN_POINT('Ctrl Pts',(-19.9254937183086,-17.2021219057221,
-19.0109264168999));
#68354=CARTESIAN_POINT('Ctrl Pts',(-19.9358248360724,-17.2092025524012,
-19.0101779871691));
#68355=CARTESIAN_POINT('Ctrl Pts',(-19.9408193670174,-17.212657337805,-19.0098159131762));
#68356=CARTESIAN_POINT('Ctrl Pts',(-19.9527192151025,-17.2209645577646,
-19.0089526065529));
#68357=CARTESIAN_POINT('Ctrl Pts',(-19.9596105511618,-17.225836911659,-19.0084521390993));
#68358=CARTESIAN_POINT('Ctrl Pts',(-19.9843472102746,-17.2435491921045,
-19.00665364209));
#68359=CARTESIAN_POINT('Ctrl Pts',(-20.0020217954633,-17.2566259737511,
-19.0053647341329));
#68360=CARTESIAN_POINT('Ctrl Pts',(-20.1679063497703,-17.3834035594385,
-18.9932203827108));
#68361=CARTESIAN_POINT('Ctrl Pts',(-20.3006543931763,-17.5159700118114,
-18.9832348475224));
#68362=CARTESIAN_POINT('Ctrl Pts',(-20.4625576818018,-17.7272251792347,
-18.9687214806273));
#68363=CARTESIAN_POINT('Ctrl Pts',(-20.5072415291622,-17.79286345203,-18.9643555453313));
#68364=CARTESIAN_POINT('Ctrl Pts',(-20.5665926695611,-17.8915398015072,
-18.9577673506855));
#68365=CARTESIAN_POINT('Ctrl Pts',(-20.5842696000682,-17.9226925680994,
-18.9556837747955));
#68366=CARTESIAN_POINT('Ctrl Pts',(-20.6046593272031,-17.9608500459633,
-18.9531090434137));
#68367=CARTESIAN_POINT('Ctrl Pts',(-20.6081371455009,-17.9674419743132,
-18.9526634411636));
#68368=CARTESIAN_POINT('Ctrl Pts',(-20.6135001060839,-17.9777384193655,
-18.9519659597463));
#68369=CARTESIAN_POINT('Ctrl Pts',(-20.6154093087419,-17.9814304308465,
-18.9517155719581));
#68370=CARTESIAN_POINT('Ctrl Pts',(-20.6189363544477,-17.9883005357199,
-18.9512490657672));
#68371=CARTESIAN_POINT('Ctrl Pts',(-20.6205570443778,-17.9914771030985,
-18.9510331299139));
#68372=CARTESIAN_POINT('Ctrl Pts',(-20.6242111984938,-17.9986842049165,
-18.9505426817761));
#68373=CARTESIAN_POINT('Ctrl Pts',(-20.6262397910603,-18.0027171378762,
-18.9502678706272));
#68374=CARTESIAN_POINT('Ctrl Pts',(-20.6322139783063,-18.0146893297531,
-18.9494510467547));
#68375=CARTESIAN_POINT('Ctrl Pts',(-20.6361225596381,-18.0226468045976,
-18.9489068120163));
#68376=CARTESIAN_POINT('Ctrl Pts',(-20.6648568493489,-18.082087546218,-18.9448329805944));
#68377=CARTESIAN_POINT('Ctrl Pts',(-20.6876362615745,-18.1345283096112,
-18.9411920412909));
#68378=CARTESIAN_POINT('Ctrl Pts',(-20.7683686241143,-18.3431011474956,
-18.9267030005516));
#68379=CARTESIAN_POINT('Ctrl Pts',(-20.809946228261,-18.5049335841527,-18.9155001551014));
#68380=CARTESIAN_POINT('Ctrl Pts',(-20.8399080681384,-18.727838418948,-18.9010061891986));
#68381=CARTESIAN_POINT('Ctrl Pts',(-20.8452891034385,-18.7859985162162,
-18.8973011530895));
#68382=CARTESIAN_POINT('Ctrl Pts',(-20.8500786755013,-18.880032259341,-18.8914414621977));
#68383=CARTESIAN_POINT('Ctrl Pts',(-20.8509926290197,-18.9157954380901,
-18.8892429548497));
#68384=CARTESIAN_POINT('Ctrl Pts',(-20.8510022031581,-18.9625398042562,
-18.8864068683001));
#68385=CARTESIAN_POINT('Ctrl Pts',(-20.850919130275,-18.9735132198352,-18.8857437716456));
#68386=CARTESIAN_POINT('Ctrl Pts',(-20.8506443290979,-18.9914191399575,
-18.8846660223645));
#68387=CARTESIAN_POINT('Ctrl Pts',(-20.8505038547557,-18.9983521205708,
-18.8842497718997));
#68388=CARTESIAN_POINT('Ctrl Pts',(-20.8501671510663,-19.0117252006668,
-18.8834488320296));
#68389=CARTESIAN_POINT('Ctrl Pts',(-20.8499755814384,-19.0181653309523,
-18.8830640011775));
#68390=CARTESIAN_POINT('Ctrl Pts',(-20.8494626513394,-19.0331125256614,
-18.882172829525));
#68391=CARTESIAN_POINT('Ctrl Pts',(-20.8491193704855,-19.0416187639829,
-18.881667180825));
#68392=CARTESIAN_POINT('Ctrl Pts',(-20.8478634330838,-19.068686500085,-18.8800627833598));
#68393=CARTESIAN_POINT('Ctrl Pts',(-20.8467576624232,-19.0872384764525,
-18.878970085231));
#68394=CARTESIAN_POINT('Ctrl Pts',(-20.8436139253888,-19.130403857889,-18.8764424037144));
#68395=CARTESIAN_POINT('Ctrl Pts',(-20.8413892477373,-19.1550011838357,
-18.8750132232758));
#68396=CARTESIAN_POINT('Ctrl Pts',(-20.8320826336087,-19.241081379516,-18.8700446278674));
#68397=CARTESIAN_POINT('Ctrl Pts',(-20.8227356923287,-19.3022896673205,
-18.8665717938389));
#68398=CARTESIAN_POINT('Ctrl Pts',(-20.7895029612841,-19.4702078065612,
-18.857102788481));
#68399=CARTESIAN_POINT('Ctrl Pts',(-20.7600278810369,-19.5755543537232,
-18.8512347937857));
#68400=CARTESIAN_POINT('Ctrl Pts',(-20.7225806288389,-19.6781102413592,
-18.845275429269));
#68401=CARTESIAN_POINT('Origin',(-18.734,-18.952,0.));
#68402=CARTESIAN_POINT('',(-20.7225806448396,-19.6781101975385,-18.0457833736847));
#68403=CARTESIAN_POINT('',(-20.7225805813239,-19.6781103714872,-18.2676550109742));
#68404=CARTESIAN_POINT('',(-20.7225805821191,-19.6781103693095,0.));
#68405=CARTESIAN_POINT('',(-20.8509999976816,-18.9519009238279,-18.3109437209775));
#68406=CARTESIAN_POINT('Ctrl Pts',(-20.7225805813239,-19.6781103714872,
-18.2676550109742));
#68407=CARTESIAN_POINT('Ctrl Pts',(-20.7255215254997,-19.6700560801449,
-18.2681338976806));
#68408=CARTESIAN_POINT('Ctrl Pts',(-20.7284136840267,-19.6619835175783,
-18.2686116714034));
#68409=CARTESIAN_POINT('Ctrl Pts',(-20.7649458433877,-19.5580302170336,
-18.2747374158079));
#68410=CARTESIAN_POINT('Ctrl Pts',(-20.7916902777909,-19.4598634697817,
-18.280222863525));
#68411=CARTESIAN_POINT('Ctrl Pts',(-20.8346520007344,-19.2412122723913,
-18.2923391376341));
#68412=CARTESIAN_POINT('Ctrl Pts',(-20.8477603784538,-19.1204977421627,
-18.2989652682401));
#68413=CARTESIAN_POINT('Ctrl Pts',(-20.8507279701885,-18.9878359543606,
-18.3067852888075));
#68414=CARTESIAN_POINT('Ctrl Pts',(-20.8508915333075,-18.9763256758259,
-18.3074682690814));
#68415=CARTESIAN_POINT('Ctrl Pts',(-20.8509827804114,-18.9612521100644,
-18.308369215915));
#68416=CARTESIAN_POINT('Ctrl Pts',(-20.8509953532782,-18.9576892778179,
-18.3085826443122));
#68417=CARTESIAN_POINT('Ctrl Pts',(-20.8509997175536,-18.9533444198951,
-18.3088435204735));
#68418=CARTESIAN_POINT('Ctrl Pts',(-20.8510000697472,-18.9525623810612,
-18.3088904997976));
#68419=CARTESIAN_POINT('Ctrl Pts',(-20.8509999886044,-18.9517803438104,
-18.3089375029375));
#68420=CARTESIAN_POINT('Ctrl Pts',(-20.8509999976816,-18.9519009238279,
-18.3109437209775));
#68421=CARTESIAN_POINT('Ctrl Pts',(-20.8509997507685,-18.9466250329455,
-18.3112630160645));
#68422=CARTESIAN_POINT('Ctrl Pts',(-20.8509797813958,-18.9413491960952,
-18.3115823111514));
#68423=CARTESIAN_POINT('Ctrl Pts',(-20.8509400905189,-18.936073507803,-18.3119016062384));
#68424=CARTESIAN_POINT('Ctrl Pts',(-20.8503946018242,-18.8635674674005,
-18.3162898151688));
#68425=CARTESIAN_POINT('Ctrl Pts',(-20.8461186979221,-18.7909479534651,
-18.3206780240991));
#68426=CARTESIAN_POINT('Ctrl Pts',(-20.8380978239802,-18.7186304494545,
-18.3250662330295));
#68427=CARTESIAN_POINT('Ctrl Pts',(-20.8300888543451,-18.6464202766104,
-18.3294479291303));
#68428=CARTESIAN_POINT('Ctrl Pts',(-20.8183460011054,-18.5745116993627,
-18.333829625231));
#68429=CARTESIAN_POINT('Ctrl Pts',(-20.8029067175878,-18.5033197197112,
-18.3382113213317));
#68430=CARTESIAN_POINT('Ctrl Pts',(-20.787485576457,-18.4322113963014,-18.3425878685909));
#68431=CARTESIAN_POINT('Ctrl Pts',(-20.7683767353657,-18.3618184668112,
-18.34696441585));
#68432=CARTESIAN_POINT('Ctrl Pts',(-20.7456691798647,-18.292548628948,-18.3513409631091));
#68433=CARTESIAN_POINT('Ctrl Pts',(-20.7229760251654,-18.2233227210093,
-18.3557147348256));
#68434=CARTESIAN_POINT('Ctrl Pts',(-20.6966888342334,-18.1552189487538,
-18.360088506542));
#68435=CARTESIAN_POINT('Ctrl Pts',(-20.66694683346,-18.0886312844346,-18.3644622782585));
#68436=CARTESIAN_POINT('Ctrl Pts',(-20.6372138832772,-18.0220638829652,
-18.3688347190215));
#68437=CARTESIAN_POINT('Ctrl Pts',(-20.6040284070361,-17.9570121136714,
-18.3732071597846));
#68438=CARTESIAN_POINT('Ctrl Pts',(-20.567577676683,-17.8938497726835,-18.3775796005476));
#68439=CARTESIAN_POINT('Ctrl Pts',(-20.5311260142806,-17.8306858166275,
-18.3819521531145));
#68440=CARTESIAN_POINT('Ctrl Pts',(-20.4914091748402,-17.7694118015958,
-18.3863247056813));
#68441=CARTESIAN_POINT('Ctrl Pts',(-20.4486594348621,-17.7103752489426,
-18.3906972582482));
#68442=CARTESIAN_POINT('Ctrl Pts',(-20.4058653275914,-17.6512774259282,
-18.395074348815));
#68443=CARTESIAN_POINT('Ctrl Pts',(-20.3600323187913,-17.5944220931037,
-18.3994514393818));
#68444=CARTESIAN_POINT('Ctrl Pts',(-20.3114344316444,-17.5401254964188,
-18.4038285299487));
#68445=CARTESIAN_POINT('Ctrl Pts',(-20.2628100033876,-17.4857992463471,
-18.4082080110071));
#68446=CARTESIAN_POINT('Ctrl Pts',(-20.2114180304778,-17.434034857225,-18.4125874920656));
#68447=CARTESIAN_POINT('Ctrl Pts',(-20.1575691237198,-17.3851113792003,
-18.416966973124));
#68448=CARTESIAN_POINT('Ctrl Pts',(-20.1036247701359,-17.3361011846391,
-18.4213542167833));
#68449=CARTESIAN_POINT('Ctrl Pts',(-20.0472151597982,-17.2899422626071,
-18.4257414604425));
#68450=CARTESIAN_POINT('Ctrl Pts',(-19.9886831896908,-17.2468727046031,
-18.4301287041018));
#68451=CARTESIAN_POINT('Ctrl Pts',(-19.9488870900799,-17.2175895552853,
-18.4331116070411));
#68452=CARTESIAN_POINT('Ctrl Pts',(-19.9081105258033,-17.1897336331323,
-18.4360945099805));
#68453=CARTESIAN_POINT('Ctrl Pts',(-19.8664678605231,-17.1633676887403,
-18.4390774129199));
#68454=CARTESIAN_POINT('Ctrl Pts',(-19.8052064921926,-17.1245802139255,
-18.4434656218502));
#68455=CARTESIAN_POINT('Ctrl Pts',(-19.7418305075797,-17.0888680068776,
-18.4478538307804));
#68456=CARTESIAN_POINT('Ctrl Pts',(-19.6766813842659,-17.0564681992226,
-18.4522420397107));
#68457=CARTESIAN_POINT('Ctrl Pts',(-19.6116289530532,-17.0241164782542,
-18.4566237358114));
#68458=CARTESIAN_POINT('Ctrl Pts',(-19.544809035632,-16.9950676104731,-18.461005431912));
#68459=CARTESIAN_POINT('Ctrl Pts',(-19.476590855784,-16.9695147362702,-18.4653871280126));
#68460=CARTESIAN_POINT('Ctrl Pts',(-19.4084528377265,-16.943991888728,-18.4697636752716));
#68461=CARTESIAN_POINT('Ctrl Pts',(-19.338920270696,-16.9219570424212,-18.4741402225306));
#68462=CARTESIAN_POINT('Ctrl Pts',(-19.2683841301356,-16.9035560536204,
-18.4785167697896));
#68463=CARTESIAN_POINT('Ctrl Pts',(-19.1978927225705,-16.8851667344593,
-18.482890541506));
#68464=CARTESIAN_POINT('Ctrl Pts',(-19.1263994698867,-16.8704068217633,
-18.4872643132223));
#68465=CARTESIAN_POINT('Ctrl Pts',(-19.0543110010062,-16.8593724978787,
-18.4916380849386));
#68466=CARTESIAN_POINT('Ctrl Pts',(-18.9822444688891,-16.848341531776,-18.4960105257015));
#68467=CARTESIAN_POINT('Ctrl Pts',(-18.9095835567044,-16.8410339766645,
-18.5003829664644));
#68468=CARTESIAN_POINT('Ctrl Pts',(-18.8367439345959,-16.8374946952292,
-18.5047554072273));
#68469=CARTESIAN_POINT('Ctrl Pts',(-18.7639024499703,-16.8339553232942,
-18.509127959794));
#68470=CARTESIAN_POINT('Ctrl Pts',(-18.6908827282545,-16.8341844377533,
-18.5135005123607));
#68471=CARTESIAN_POINT('Ctrl Pts',(-18.6181027067752,-16.8381748375461,
-18.5178730649274));
#68472=CARTESIAN_POINT('Ctrl Pts',(-18.5452471514446,-16.8421693787263,
-18.5222501554941));
#68473=CARTESIAN_POINT('Ctrl Pts',(-18.4726322757212,-16.8499329725835,
-18.5266272460608));
#68474=CARTESIAN_POINT('Ctrl Pts',(-18.4006723159531,-16.8614063869207,
-18.5310043366275));
#68475=CARTESIAN_POINT('Ctrl Pts',(-18.3286730561801,-16.8728860673153,
-18.5353838176857));
#68476=CARTESIAN_POINT('Ctrl Pts',(-18.2573298966123,-16.8880795015318,
-18.539763298744));
#68477=CARTESIAN_POINT('Ctrl Pts',(-18.1870456020006,-16.9068765595913,
-18.5441427798023));
#68478=CARTESIAN_POINT('Ctrl Pts',(-18.1166367289484,-16.92570693531,-18.5485300234614));
#68479=CARTESIAN_POINT('Ctrl Pts',(-18.0472909281459,-16.9481535415646,
-18.5529172671205));
#68480=CARTESIAN_POINT('Ctrl Pts',(-17.9793940004985,-16.9740569306685,
-18.5573045107795));
#68481=CARTESIAN_POINT('Ctrl Pts',(-17.9332306321349,-16.9916687392511,
-18.5602874137201));
#68482=CARTESIAN_POINT('Ctrl Pts',(-17.8877366290263,-17.0108774944519,
-18.5632703166607));
#68483=CARTESIAN_POINT('Ctrl Pts',(-17.8430266573748,-17.0316210002369,
-18.5662532196012));
#68484=CARTESIAN_POINT('Ctrl Pts',(-17.7772529124845,-17.0621371917538,
-18.5706414285354));
#68485=CARTESIAN_POINT('Ctrl Pts',(-17.7129203794319,-17.0960960250395,
-18.5750296374695));
#68486=CARTESIAN_POINT('Ctrl Pts',(-17.6504132837262,-17.1333387263388,
-18.5794178464036));
#68487=CARTESIAN_POINT('Ctrl Pts',(-17.5879989589142,-17.1705261532945,
-18.5837995425081));
#68488=CARTESIAN_POINT('Ctrl Pts',(-17.5274051041878,-17.2109875282323,
-18.5881812386126));
#68489=CARTESIAN_POINT('Ctrl Pts',(-17.4689939738811,-17.2545169356124,
-18.5925629347171));
#68490=CARTESIAN_POINT('Ctrl Pts',(-17.410651481301,-17.2979951924746,-18.59693948198));
#68491=CARTESIAN_POINT('Ctrl Pts',(-17.3544870028672,-17.3445340332485,
-18.6013160292429));
#68492=CARTESIAN_POINT('Ctrl Pts',(-17.3008348082133,-17.393883658692,-18.6056925765057));
#68493=CARTESIAN_POINT('Ctrl Pts',(-17.2472166390015,-17.4432019873203,
-18.6100663482259));
#68494=CARTESIAN_POINT('Ctrl Pts',(-17.1961079465048,-17.4953272380339,
-18.6144401199461));
#68495=CARTESIAN_POINT('Ctrl Pts',(-17.1478097053788,-17.5499695619391,
-18.6188138916663));
#68496=CARTESIAN_POINT('Ctrl Pts',(-17.0995261615698,-17.6045952580014,
-18.6231863324331));
#68497=CARTESIAN_POINT('Ctrl Pts',(-17.0540516905101,-17.6617361453902,
-18.6275587731999));
#68498=CARTESIAN_POINT('Ctrl Pts',(-17.0116490089833,-17.7210669946159,
-18.6319312139666));
#68499=CARTESIAN_POINT('Ctrl Pts',(-16.9692452432155,-17.7803993609378,
-18.6363037665372));
#68500=CARTESIAN_POINT('Ctrl Pts',(-16.9299137017786,-17.8419214066584,
-18.6406763191077));
#68501=CARTESIAN_POINT('Ctrl Pts',(-16.8938745512688,-17.9052778148278,
-18.6450488716783));
#68502=CARTESIAN_POINT('Ctrl Pts',(-16.8577979979695,-17.9686999766668,
-18.6494259622488));
#68503=CARTESIAN_POINT('Ctrl Pts',(-16.8250208968186,-18.0339598817744,
-18.6538030528193));
#68504=CARTESIAN_POINT('Ctrl Pts',(-16.7957176611908,-18.1006771616711,
-18.6581801433897));
#68505=CARTESIAN_POINT('Ctrl Pts',(-16.7663984219786,-18.1674308783503,
-18.6625596244518));
#68506=CARTESIAN_POINT('Ctrl Pts',(-16.7405569966195,-18.2356431030953,
-18.6669391055139));
#68507=CARTESIAN_POINT('Ctrl Pts',(-16.7183187921507,-18.3049155632198,
-18.671318586576));
#68508=CARTESIAN_POINT('Ctrl Pts',(-16.6960411706141,-18.3743108083137,
-18.6757058302388));
#68509=CARTESIAN_POINT('Ctrl Pts',(-16.6773796475295,-18.444769574883,-18.6800930739016));
#68510=CARTESIAN_POINT('Ctrl Pts',(-16.662408979339,-18.5158811594111,-18.6844803175644));
#68511=CARTESIAN_POINT('Ctrl Pts',(-16.6522303676447,-18.5642301840949,
-18.6874632204705));
#68512=CARTESIAN_POINT('Ctrl Pts',(-16.6437568500116,-18.6128807754369,
-18.6904461233766));
#68513=CARTESIAN_POINT('Ctrl Pts',(-16.6369981960583,-18.6617028517788,
-18.6934290262827));
#68514=CARTESIAN_POINT('Ctrl Pts',(-16.6270554032346,-18.7335259978735,
-18.6978172352091));
#68515=CARTESIAN_POINT('Ctrl Pts',(-16.6207874279489,-18.8060007495847,
-18.7022054441356));
#68516=CARTESIAN_POINT('Ctrl Pts',(-16.6182687405808,-18.8787180928431,
-18.706593653062));
#68517=CARTESIAN_POINT('Ctrl Pts',(-16.6157537913624,-18.9513275115075,
-18.7109753491589));
#68518=CARTESIAN_POINT('Ctrl Pts',(-16.6169771002007,-19.0241783288748,
-18.7153570452557));
#68519=CARTESIAN_POINT('Ctrl Pts',(-16.6219616061143,-19.0968544882031,
-18.7197387413525));
#68520=CARTESIAN_POINT('Ctrl Pts',(-16.6269402548368,-19.169445247261,-18.7241152886078));
#68521=CARTESIAN_POINT('Ctrl Pts',(-16.6356712880178,-19.241861277126,-18.728491835863));
#68522=CARTESIAN_POINT('Ctrl Pts',(-16.6481255978392,-19.3136862983448,
-18.7328683831182));
#68523=CARTESIAN_POINT('Ctrl Pts',(-16.6605720093185,-19.3854657691794,
-18.7372421548308));
#68524=CARTESIAN_POINT('Ctrl Pts',(-16.6767369302053,-19.4566545009215,
-18.7416159265435));
#68525=CARTESIAN_POINT('Ctrl Pts',(-16.6965395553228,-19.5268425318082,
-18.7459896982561));
#68526=CARTESIAN_POINT('Ctrl Pts',(-16.716336154435,-19.5970092042419,-18.7503621390153));
#68527=CARTESIAN_POINT('Ctrl Pts',(-16.7397681292056,-19.6661753164048,
-18.7547345797745));
#68528=CARTESIAN_POINT('Ctrl Pts',(-16.7667042167151,-19.7339439245044,
-18.7591070205337));
#68529=CARTESIAN_POINT('Ctrl Pts',(-16.7936409929835,-19.8017142654554,
-18.7634795730968));
#68530=CARTESIAN_POINT('Ctrl Pts',(-16.8240818798531,-19.8680865838683,
-18.7678521256598));
#68531=CARTESIAN_POINT('Ctrl Pts',(-16.8578472840023,-19.9326834281533,
-18.7722246782229));
#68532=CARTESIAN_POINT('Ctrl Pts',(-16.8916477311622,-19.9973473134812,
-18.776601768786));
#68533=CARTESIAN_POINT('Ctrl Pts',(-16.9287793604415,-20.060231617285,-18.7809788593491));
#68534=CARTESIAN_POINT('Ctrl Pts',(-16.9690167487956,-20.1209837992753,
-18.7853559499122));
#68535=CARTESIAN_POINT('Ctrl Pts',(-17.0092761122814,-20.1817691602876,
-18.789735430967));
#68536=CARTESIAN_POINT('Ctrl Pts',(-17.0526443249046,-20.240419692987,-18.7941149120218));
#68537=CARTESIAN_POINT('Ctrl Pts',(-17.0988543828153,-20.296614372451,-18.7984943930766));
#68538=CARTESIAN_POINT('Ctrl Pts',(-17.1451463477448,-20.3529086566087,
-18.8028816367322));
#68539=CARTESIAN_POINT('Ctrl Pts',(-17.1942898914284,-20.4067380382408,
-18.8072688803879));
#68540=CARTESIAN_POINT('Ctrl Pts',(-17.245980141449,-20.4578173529873,-18.8116561240436));
#68541=CARTESIAN_POINT('Ctrl Pts',(-17.2811245310909,-20.4925463655067,
-18.8146390270171));
#68542=CARTESIAN_POINT('Ctrl Pts',(-17.3174454256977,-20.5260048960133,
-18.8176219299906));
#68543=CARTESIAN_POINT('Ctrl Pts',(-17.3548387352824,-20.5581143190641,
-18.8206048329642));
#68544=CARTESIAN_POINT('Ctrl Pts',(-17.4098487897263,-20.6053511411,-18.8249930418924));
#68545=CARTESIAN_POINT('Ctrl Pts',(-17.4673958504111,-20.6498507248998,
-18.8293812508206));
#68546=CARTESIAN_POINT('Ctrl Pts',(-17.5271763106365,-20.6913290611011,
-18.8337694597488));
#68547=CARTESIAN_POINT('Ctrl Pts',(-17.5868680467462,-20.7327458365737,
-18.8381511558473));
#68548=CARTESIAN_POINT('Ctrl Pts',(-17.6487862091488,-20.7711499931513,
-18.8425328519459));
#68549=CARTESIAN_POINT('Ctrl Pts',(-17.7125933764222,-20.806297039126,-18.8469145480444));
#68550=CARTESIAN_POINT('Ctrl Pts',(-17.776325565195,-20.8414027845239,-18.8512910953012));
#68551=CARTESIAN_POINT('Ctrl Pts',(-17.8419419289072,-20.873258790821,-18.855667642558));
#68552=CARTESIAN_POINT('Ctrl Pts',(-17.9090766869063,-20.9016642089125,
-18.8600441898149));
#68553=CARTESIAN_POINT('Ctrl Pts',(-17.9761688690169,-20.9300516127005,
-18.864417961529));
#68554=CARTESIAN_POINT('Ctrl Pts',(-18.0447770916536,-20.9549925826758,
-18.8687917332431));
#68555=CARTESIAN_POINT('Ctrl Pts',(-18.114512903542,-20.9763331586777,-18.8731655049572));
#68556=CARTESIAN_POINT('Ctrl Pts',(-18.184227494588,-20.9976672406704,-18.8775379457179));
#68557=CARTESIAN_POINT('Ctrl Pts',(-18.255068532683,-21.0154029627463,-18.8819103864785));
#68558=CARTESIAN_POINT('Ctrl Pts',(-18.3266312007864,-21.0294358381012,
-18.8862828272392));
#68559=CARTESIAN_POINT('Ctrl Pts',(-18.3981956987546,-21.0434690722781,
-18.8906553798036));
#68560=CARTESIAN_POINT('Ctrl Pts',(-18.4704813896189,-21.0537991808911,
-18.895027932368));
#68561=CARTESIAN_POINT('Ctrl Pts',(-18.5430736858662,-21.0603728661153,
-18.8994004849324));
#68562=CARTESIAN_POINT('Ctrl Pts',(-18.6157413211363,-21.0669533737579,
-18.9037775754968));
#68563=CARTESIAN_POINT('Ctrl Pts',(-18.6887157156707,-21.0697696306808,
-18.9081546660611));
#68564=CARTESIAN_POINT('Ctrl Pts',(-18.7615784216581,-21.0688203586178,
-18.9125317566255));
#68565=CARTESIAN_POINT('Ctrl Pts',(-18.8344809206732,-21.0678705681221,
-18.9169112376815));
#68566=CARTESIAN_POINT('Ctrl Pts',(-18.9072711279956,-21.0631511854102,
-18.9212907187374));
#68567=CARTESIAN_POINT('Ctrl Pts',(-18.9795345883492,-21.0547129537634,
-18.9256701997934));
#68568=CARTESIAN_POINT('Ctrl Pts',(-19.0519261352012,-21.0462597654076,
-18.9300574434501));
#68569=CARTESIAN_POINT('Ctrl Pts',(-19.123788594604,-21.0340746456029,-18.9344446871069));
#68570=CARTESIAN_POINT('Ctrl Pts',(-19.1947171668018,-21.0182595897452,
-18.9388319307636));
#68571=CARTESIAN_POINT('Ctrl Pts',(-19.2429417616859,-21.0075068755967,
-18.9418148337242));
#68572=CARTESIAN_POINT('Ctrl Pts',(-19.2907349020827,-20.9950772191557,
-18.9447977366849));
#68573=CARTESIAN_POINT('Ctrl Pts',(-19.3379741345032,-20.9810155851671,
-18.9477806396456));
#68574=CARTESIAN_POINT('Ctrl Pts',(-19.4074719557487,-20.9603282692375,
-18.9521690525416));
#68575=CARTESIAN_POINT('Ctrl Pts',(-19.4760413397801,-20.9360257809649,
-18.9565574654376));
#68576=CARTESIAN_POINT('Ctrl Pts',(-19.5432790871468,-20.9082096920082,
-18.9609458783336));
#68577=CARTESIAN_POINT('Ctrl Pts',(-19.6105530555228,-20.8803786185101,
-18.96533665527));
#68578=CARTESIAN_POINT('Ctrl Pts',(-19.6764934757503,-20.849030254655,-18.9697274322063));
#68579=CARTESIAN_POINT('Ctrl Pts',(-19.7407097293466,-20.8143169764675,
-18.9741182091426));
#68580=CARTESIAN_POINT('Ctrl Pts',(-19.8047168405566,-20.7797167540474,
-18.9784946859989));
#68581=CARTESIAN_POINT('Ctrl Pts',(-19.8670105560363,-20.741773696628,-18.9828711628552));
#68582=CARTESIAN_POINT('Ctrl Pts',(-19.9272240703357,-20.7006867409492,
-18.9872476397115));
#68583=CARTESIAN_POINT('Ctrl Pts',(-19.987398312053,-20.6596265830891,-18.991621262133));
#68584=CARTESIAN_POINT('Ctrl Pts',(-20.0454946477979,-20.6154268676538,
-18.9959948845546));
#68585=CARTESIAN_POINT('Ctrl Pts',(-20.1011734566812,-20.5683309498201,
-19.0003685069761));
#68586=CARTESIAN_POINT('Ctrl Pts',(-20.1568343181235,-20.5212502128284,
-19.0047407196094));
#68587=CARTESIAN_POINT('Ctrl Pts',(-20.2100788325333,-20.4712754389994,
-19.0091129322427));
#68588=CARTESIAN_POINT('Ctrl Pts',(-20.2606001433951,-20.418690492976,-19.0134851448761));
#68589=CARTESIAN_POINT('Ctrl Pts',(-20.3114804596682,-20.36573187731,-19.0178884265368));
#68590=CARTESIAN_POINT('Ctrl Pts',(-20.3595983474391,-20.3101261777265,
-19.0222917081976));
#68591=CARTESIAN_POINT('Ctrl Pts',(-20.4046790961748,-20.2522001221368,
-19.0266949898584));
#68592=CARTESIAN_POINT('Ctrl Pts',(-20.4494793719813,-20.1946344574222,
-19.0310708762043));
#68593=CARTESIAN_POINT('Ctrl Pts',(-20.4912799489289,-20.1347776523353,
-19.0354467625502));
#68594=CARTESIAN_POINT('Ctrl Pts',(-20.5298538380763,-20.0729808170823,
-19.0398226488961));
#68595=CARTESIAN_POINT('Ctrl Pts',(-20.5687899660098,-20.0106036615382,
-19.0442396282143));
#68596=CARTESIAN_POINT('Ctrl Pts',(-20.6044382264007,-19.9462502770228,
-19.0486566075325));
#68597=CARTESIAN_POINT('Ctrl Pts',(-20.6366128839545,-19.8803066378144,
-19.0530735868507));
#68598=CARTESIAN_POINT('Ctrl Pts',(-20.6687875415084,-19.8143629986061,
-19.0574905661689));
#68599=CARTESIAN_POINT('Ctrl Pts',(-20.6974884458848,-19.7468295847188,
-19.0619075454871));
#68600=CARTESIAN_POINT('Ctrl Pts',(-20.7225805821191,-19.6781103693095,
-19.0663245248053));
#68601=CARTESIAN_POINT('',(-20.8509990913815,-18.9539458517612,-18.0890147820491));
#68602=CARTESIAN_POINT('Ctrl Pts',(-20.7225806288389,-19.6781102413592,
-18.845275429269));
#68603=CARTESIAN_POINT('Ctrl Pts',(-20.7113120014844,-19.7089713596775,
-18.8434821372632));
#68604=CARTESIAN_POINT('Ctrl Pts',(-20.6993214725324,-19.7395797295342,
-18.8416797662662));
#68605=CARTESIAN_POINT('Ctrl Pts',(-20.657531029883,-19.8393471149109,-18.8356908521596));
#68606=CARTESIAN_POINT('Ctrl Pts',(-20.6247651395845,-19.9071759854405,
-18.831436247592));
#68607=CARTESIAN_POINT('Ctrl Pts',(-20.5838855794443,-19.9814184507202,
-18.8264131589613));
#68608=CARTESIAN_POINT('Ctrl Pts',(-20.5792539165066,-19.9896979231735,
-18.8258476608105));
#68609=CARTESIAN_POINT('Ctrl Pts',(-20.5723045560486,-20.0019268191934,
-18.8250040650667));
#68610=CARTESIAN_POINT('Ctrl Pts',(-20.5700293673794,-20.0059004353672,
-18.8247286333159));
#68611=CARTESIAN_POINT('Ctrl Pts',(-20.5659565592962,-20.012960377082,-18.8242368678269));
#68612=CARTESIAN_POINT('Ctrl Pts',(-20.5641640033352,-20.0160495653639,
-18.8240208624185));
#68613=CARTESIAN_POINT('Ctrl Pts',(-20.5602911303876,-20.0226851128661,
-18.8235550902555));
#68614=CARTESIAN_POINT('Ctrl Pts',(-20.5582083279712,-20.0262299005994,
-18.8233051674174));
#68615=CARTESIAN_POINT('Ctrl Pts',(-20.552425525058,-20.0360065202143,-18.8226128731409));
#68616=CARTESIAN_POINT('Ctrl Pts',(-20.5487038691006,-20.042225384965,-18.8221691273205));
#68617=CARTESIAN_POINT('Ctrl Pts',(-20.5280540936028,-20.0763323439591,
-18.8197173080956));
#68618=CARTESIAN_POINT('Ctrl Pts',(-20.5105159779353,-20.1038437478274,
-18.8176726958952));
#68619=CARTESIAN_POINT('Ctrl Pts',(-20.4017833033109,-20.2660153666386,
-18.8052648011962));
#68620=CARTESIAN_POINT('Ctrl Pts',(-20.2959558676007,-20.3902042065759,
-18.7943130197274));
#68621=CARTESIAN_POINT('Ctrl Pts',(-20.0915015931583,-20.5806550692884,
-18.7760619429663));
#68622=CARTESIAN_POINT('Ctrl Pts',(-19.9995962833844,-20.6530590110026,
-18.7686228267474));
#68623=CARTESIAN_POINT('Ctrl Pts',(-19.8902556562268,-20.7254052083604,
-18.7606173743255));
#68624=CARTESIAN_POINT('Ctrl Pts',(-19.8782592711468,-20.7331692540876,
-18.7597494193885));
#68625=CARTESIAN_POINT('Ctrl Pts',(-19.8590411958269,-20.7453328706065,
-18.7583751378124));
#68626=CARTESIAN_POINT('Ctrl Pts',(-19.8518703300315,-20.7498115600863,
-18.7578658832841));
#68627=CARTESIAN_POINT('Ctrl Pts',(-19.8391760167595,-20.7576346975449,
-18.7569705122325));
#68628=CARTESIAN_POINT('Ctrl Pts',(-19.833663773786,-20.7609970356675,-18.756583739615));
#68629=CARTESIAN_POINT('Ctrl Pts',(-19.8222308215271,-20.7678992986477,
-18.7557856695663));
#68630=CARTESIAN_POINT('Ctrl Pts',(-19.8163080136316,-20.7714356127963,
-18.7553745075329));
#68631=CARTESIAN_POINT('Ctrl Pts',(-19.80106051524,-20.7804385928158,-18.7543217847417));
#68632=CARTESIAN_POINT('Ctrl Pts',(-19.7917109782977,-20.7858629512126,
-18.7536817653604));
#68633=CARTESIAN_POINT('Ctrl Pts',(-19.7525150524015,-20.8082039324084,
-18.7510209970589));
#68634=CARTESIAN_POINT('Ctrl Pts',(-19.7223002406934,-20.8244659627158,
-18.7490237792016));
#68635=CARTESIAN_POINT('Ctrl Pts',(-19.6425552346503,-20.8649174921721,
-18.7438794181247));
#68636=CARTESIAN_POINT('Ctrl Pts',(-19.5924513304059,-20.887920428399,-18.7407716695933));
#68637=CARTESIAN_POINT('Ctrl Pts',(-19.4404220406322,-20.9506530887483,
-18.7316269284304));
#68638=CARTESIAN_POINT('Ctrl Pts',(-19.3362576097056,-20.9844696611473,
-18.7257386640872));
#68639=CARTESIAN_POINT('Ctrl Pts',(-19.1852142672726,-21.0208673072533,
-18.7172798235204));
#68640=CARTESIAN_POINT('Ctrl Pts',(-19.1401428396125,-21.030185266342,-18.714763825996));
#68641=CARTESIAN_POINT('Ctrl Pts',(-19.0730020841226,-21.0417981189295,
-18.7109848868922));
#68642=CARTESIAN_POINT('Ctrl Pts',(-19.0511418440706,-21.0452270766129,
-18.7097496572829));
#68643=CARTESIAN_POINT('Ctrl Pts',(-18.9782520515958,-21.0554924490003,
-18.7056034796288));
#68644=CARTESIAN_POINT('Ctrl Pts',(-18.9270310870913,-21.0608095271028,
-18.7026453572159));
#68645=CARTESIAN_POINT('Ctrl Pts',(-18.8670519165732,-21.0648324182433,
-18.6990774396262));
#68646=CARTESIAN_POINT('Ctrl Pts',(-18.8584285431047,-21.0653577955407,
-18.6985619652811));
#68647=CARTESIAN_POINT('Ctrl Pts',(-18.8453432492029,-21.0660746496338,
-18.697775650207));
#68648=CARTESIAN_POINT('Ctrl Pts',(-18.8408834209665,-21.0663048211763,
-18.6975069263177));
#68649=CARTESIAN_POINT('Ctrl Pts',(-18.8328642341613,-21.0666932537225,
-18.6970223773891));
#68650=CARTESIAN_POINT('Ctrl Pts',(-18.829305178454,-21.0668566421357,-18.6968068425429));
#68651=CARTESIAN_POINT('Ctrl Pts',(-18.8215561841759,-21.0671927807098,
-18.6963365033543));
#68652=CARTESIAN_POINT('Ctrl Pts',(-18.817366193203,-21.0673620640641,-18.696081512834));
#68653=CARTESIAN_POINT('Ctrl Pts',(-18.8055578732189,-21.0678040042509,
-18.695361054302));
#68654=CARTESIAN_POINT('Ctrl Pts',(-18.7979386252067,-21.0680479582875,
-18.6948940263355));
#68655=CARTESIAN_POINT('Ctrl Pts',(-18.7515931440459,-21.0692813194536,
-18.6920408113324));
#68656=CARTESIAN_POINT('Ctrl Pts',(-18.7128496717674,-21.0692486698572,
-18.6896029164142));
#68657=CARTESIAN_POINT('Ctrl Pts',(-18.5834887913314,-21.0655889202006,
-18.6813341067842));
#68658=CARTESIAN_POINT('Ctrl Pts',(-18.4931095474332,-21.0572034424621,
-18.675349326038));
#68659=CARTESIAN_POINT('Ctrl Pts',(-18.3372563683629,-21.0325740657137,
-18.6649223481402));
#68660=CARTESIAN_POINT('Ctrl Pts',(-18.2714938439103,-21.0189500604532,
-18.660487904005));
#68661=CARTESIAN_POINT('Ctrl Pts',(-18.0953526853012,-20.9736298699137,
-18.648616843998));
#68662=CARTESIAN_POINT('Ctrl Pts',(-17.9867127657187,-20.9360430775046,
-18.6413129705392));
#68663=CARTESIAN_POINT('Ctrl Pts',(-17.8685879973835,-20.8840855037306,
-18.6334336929697));
#68664=CARTESIAN_POINT('Ctrl Pts',(-17.8555936246965,-20.8782124969595,
-18.6325675657634));
#68665=CARTESIAN_POINT('Ctrl Pts',(-17.8349986264041,-20.8686525146428,
-18.631195622191));
#68666=CARTESIAN_POINT('Ctrl Pts',(-17.8273591882732,-20.8650506457892,
-18.6306868934148));
#68667=CARTESIAN_POINT('Ctrl Pts',(-17.813919146972,-20.8586152980352,-18.6297921337245));
#68668=CARTESIAN_POINT('Ctrl Pts',(-17.8081096039757,-20.8558008422081,
-18.6294054495358));
#68669=CARTESIAN_POINT('Ctrl Pts',(-17.7961156771543,-20.8499224507735,
-18.6286072618506));
#68670=CARTESIAN_POINT('Ctrl Pts',(-17.7899332142322,-20.8468547537831,
-18.6281958952319));
#68671=CARTESIAN_POINT('Ctrl Pts',(-17.7740927191565,-20.8388980335203,
-18.6271420265877));
#68672=CARTESIAN_POINT('Ctrl Pts',(-17.7644569079766,-20.8339650304978,
-18.6265010725312));
#68673=CARTESIAN_POINT('Ctrl Pts',(-17.7243188539029,-20.8130264692688,
-18.6238312039699));
#68674=CARTESIAN_POINT('Ctrl Pts',(-17.6941707057632,-20.796351044109,-18.6218260264653));
#68675=CARTESIAN_POINT('Ctrl Pts',(-17.616617273751,-20.7509485536852,-18.6166565084999));
#68676=CARTESIAN_POINT('Ctrl Pts',(-17.5699085705251,-20.7210822067612,
-18.6135320699503));
#68677=CARTESIAN_POINT('Ctrl Pts',(-17.434470496904,-20.6267911356964,-18.6043582237157));
#68678=CARTESIAN_POINT('Ctrl Pts',(-17.3495148293822,-20.5572737907738,
-18.5984574440118));
#68679=CARTESIAN_POINT('Ctrl Pts',(-17.2253041719961,-20.4384080444049,
-18.5890958148823));
#68680=CARTESIAN_POINT('Ctrl Pts',(-17.1822100864807,-20.3933602271417,
-18.585682958005));
#68681=CARTESIAN_POINT('Ctrl Pts',(-17.104104148923,-20.304144414272,-18.5790303522828));
#68682=CARTESIAN_POINT('Ctrl Pts',(-17.0687465329632,-20.2603519082761,
-18.5758083529987));
#68683=CARTESIAN_POINT('Ctrl Pts',(-17.0299078677744,-20.2081198272265,
-18.5719466220178));
#68684=CARTESIAN_POINT('Ctrl Pts',(-17.0246819733804,-20.200999156603,-18.5714197689891));
#68685=CARTESIAN_POINT('Ctrl Pts',(-17.0168568449586,-20.1901957443923,
-18.5706194961107));
#68686=CARTESIAN_POINT('Ctrl Pts',(-17.0142244882095,-20.1865369595597,
-18.570348307424));
#68687=CARTESIAN_POINT('Ctrl Pts',(-17.0095307140478,-20.1799688089324,
-18.569861135059));
#68688=CARTESIAN_POINT('Ctrl Pts',(-17.0074649452116,-20.1770626180777,
-18.5696454556193));
#68689=CARTESIAN_POINT('Ctrl Pts',(-17.003003953687,-20.1707530542269,-18.5691769229234));
#68690=CARTESIAN_POINT('Ctrl Pts',(-17.0006114540789,-20.1673478793003,
-18.5689238950526));
#68691=CARTESIAN_POINT('Ctrl Pts',(-16.993948598028,-20.1578051353874,-18.568214386248));
#68692=CARTESIAN_POINT('Ctrl Pts',(-16.9897007434413,-20.1516520352862,
-18.5677564187599));
#68693=CARTESIAN_POINT('Ctrl Pts',(-16.9650726556814,-20.1155704208854,
-18.5650687277761));
#68694=CARTESIAN_POINT('Ctrl Pts',(-16.9454316630597,-20.0851473932677,
-18.5627938810971));
#68695=CARTESIAN_POINT('Ctrl Pts',(-16.8845095968982,-19.9852491355776,
-18.555333839777));
#68696=CARTESIAN_POINT('Ctrl Pts',(-16.8464245338091,-19.9139124956362,
-18.5500237818227));
#68697=CARTESIAN_POINT('Ctrl Pts',(-16.7350527949056,-19.6730792752924,
-18.5325039700128));
#68698=CARTESIAN_POINT('Ctrl Pts',(-16.6798106516438,-19.4961310049149,
-18.5203486591922));
#68699=CARTESIAN_POINT('Ctrl Pts',(-16.6444211093995,-19.2923560817245,
-18.507628026634));
#68700=CARTESIAN_POINT('Ctrl Pts',(-16.6409655354423,-19.2704163807884,
-18.5062729822592));
#68701=CARTESIAN_POINT('Ctrl Pts',(-16.6366690847654,-19.2400344645843,
-18.5044159417195));
#68702=CARTESIAN_POINT('Ctrl Pts',(-16.6355328265435,-19.2316360956322,
-18.5039046447781));
#68703=CARTESIAN_POINT('Ctrl Pts',(-16.6336677699776,-19.2171990121298,
-18.5030291452845));
#68704=CARTESIAN_POINT('Ctrl Pts',(-16.6329145149182,-19.211163612579,-18.5026641739058));
#68705=CARTESIAN_POINT('Ctrl Pts',(-16.6314164406909,-19.198724416687,-18.5019140428557));
#68706=CARTESIAN_POINT('Ctrl Pts',(-16.6306748418307,-19.1923202906492,
-18.5015289884933));
#68707=CARTESIAN_POINT('Ctrl Pts',(-16.629019016596,-19.1774262016551,-18.5006360669791));
#68708=CARTESIAN_POINT('Ctrl Pts',(-16.6281268752855,-19.1689338580068,
-18.5001289006083));
#68709=CARTESIAN_POINT('Ctrl Pts',(-16.6254426100705,-19.1418033628106,
-18.498514751802));
#68710=CARTESIAN_POINT('Ctrl Pts',(-16.6238463273348,-19.1231464117051,
-18.4974139260147));
#68711=CARTESIAN_POINT('Ctrl Pts',(-16.6207021656623,-19.0796041267272,
-18.4948646782173));
#68712=CARTESIAN_POINT('Ctrl Pts',(-16.6193459403488,-19.0547075029223,
-18.4934221991562));
#68713=CARTESIAN_POINT('Ctrl Pts',(-16.6161240824696,-18.9670883485719,
-18.4883922207389));
#68714=CARTESIAN_POINT('Ctrl Pts',(-16.6166071118363,-18.904310285101,-18.4848732209941));
#68715=CARTESIAN_POINT('Ctrl Pts',(-16.6251112675776,-18.7413959343469,
-18.4758544023313));
#68716=CARTESIAN_POINT('Ctrl Pts',(-16.6374678711437,-18.6416465530865,
-18.4704480962761));
#68717=CARTESIAN_POINT('Ctrl Pts',(-16.6712069353561,-18.4702362445365,
-18.4609310074807));
#68718=CARTESIAN_POINT('Ctrl Pts',(-16.6893873909543,-18.3981323554564,
-18.4568528280256));
#68719=CARTESIAN_POINT('Ctrl Pts',(-16.7240800811799,-18.2858318337492,
-18.4501826082381));
#68720=CARTESIAN_POINT('Ctrl Pts',(-16.7381023266811,-18.2449285683577,
-18.4476835083764));
#68721=CARTESIAN_POINT('Ctrl Pts',(-16.756014289516,-18.1974684920272,-18.4446701367022));
#68722=CARTESIAN_POINT('Ctrl Pts',(-16.7587001891292,-18.1904647606305,
-18.4442224990094));
#68723=CARTESIAN_POINT('Ctrl Pts',(-16.7631007724207,-18.1791697540896,
-18.4434955822653));
#68724=CARTESIAN_POINT('Ctrl Pts',(-16.7647924122323,-18.1748694899721,
-18.443217650574));
#68725=CARTESIAN_POINT('Ctrl Pts',(-16.7678180275156,-18.1672514810208,
-18.4427231382059));
#68726=CARTESIAN_POINT('Ctrl Pts',(-16.7691463436995,-18.1639315409957,
-18.442506900023));
#68727=CARTESIAN_POINT('Ctrl Pts',(-16.7720098480995,-18.1568268588732,
-18.4420425691746));
#68728=CARTESIAN_POINT('Ctrl Pts',(-16.7735475558735,-18.1530432463576,
-18.4417943306171));
#68729=CARTESIAN_POINT('Ctrl Pts',(-16.7777974175703,-18.1426723750164,
-18.4411113243718));
#68730=CARTESIAN_POINT('Ctrl Pts',(-16.7805318585027,-18.1360943897149,
-18.4406752412043));
#68731=CARTESIAN_POINT('Ctrl Pts',(-16.7952897290834,-18.1010922591209,
-18.4383399539933));
#68732=CARTESIAN_POINT('Ctrl Pts',(-16.8078997887866,-18.072921367308,-18.4364081065725));
#68733=CARTESIAN_POINT('Ctrl Pts',(-16.8478987707588,-17.9885592467277,
-18.4304848560207));
#68734=CARTESIAN_POINT('Ctrl Pts',(-16.8771637006213,-17.9332979839508,
-18.4264164714451));
#68735=CARTESIAN_POINT('Ctrl Pts',(-16.9237407496424,-17.8540397004061,
-18.4203757142423));
#68736=CARTESIAN_POINT('Ctrl Pts',(-16.9391811343044,-17.8289770377254,
-18.4184335686013));
#68737=CARTESIAN_POINT('Ctrl Pts',(-17.0519720908878,-17.6541667271171,
-18.4046906165094));
#68738=CARTESIAN_POINT('Ctrl Pts',(-17.167429798326,-17.5169140828983,-18.3929511552596));
#68739=CARTESIAN_POINT('Ctrl Pts',(-17.3154944095117,-17.3803613025191,
-18.3805564180322));
#68740=CARTESIAN_POINT('Ctrl Pts',(-17.3324618116889,-17.365211710495,-18.379168173424));
#68741=CARTESIAN_POINT('Ctrl Pts',(-17.3568622310037,-17.3441222307585,
-18.3772159864981));
#68742=CARTESIAN_POINT('Ctrl Pts',(-17.364095737645,-17.337954872933,-18.3766426264557));
#68743=CARTESIAN_POINT('Ctrl Pts',(-17.375931476834,-17.3280004921146,-18.3757130708945));
#68744=CARTESIAN_POINT('Ctrl Pts',(-17.3805085345386,-17.3241838650271,
-18.3753556629683));
#68745=CARTESIAN_POINT('Ctrl Pts',(-17.3901352674176,-17.3162251882643,
-18.3746082251605));
#68746=CARTESIAN_POINT('Ctrl Pts',(-17.3951881235144,-17.3120870708959,
-18.3742183576119));
#68747=CARTESIAN_POINT('Ctrl Pts',(-17.4072768174534,-17.302279952568,-18.3732913778916));
#68748=CARTESIAN_POINT('Ctrl Pts',(-17.4143299943915,-17.2966324522461,
-18.3727551359065));
#68749=CARTESIAN_POINT('Ctrl Pts',(-17.4383218841956,-17.2776728695598,
-18.3709463729434));
#68750=CARTESIAN_POINT('Ctrl Pts',(-17.4554279173697,-17.2645739721611,
-18.3696823296548));
#68751=CARTESIAN_POINT('Ctrl Pts',(-17.5503688680766,-17.1941459748197,
-18.3627999857183));
#68752=CARTESIAN_POINT('Ctrl Pts',(-17.6318643975335,-17.1419354394404,
-18.3573829234189));
#68753=CARTESIAN_POINT('Ctrl Pts',(-17.8504842710984,-17.0221350728713,
-18.3436780779384));
#68754=CARTESIAN_POINT('Ctrl Pts',(-17.9918426882678,-16.9634893468507,
-18.3356006764855));
#68755=CARTESIAN_POINT('Ctrl Pts',(-18.1878327932578,-16.9060140012061,
-18.3240979319656));
#68756=CARTESIAN_POINT('Ctrl Pts',(-18.2379123479768,-16.8932981195625,
-18.3211302723438));
#68757=CARTESIAN_POINT('Ctrl Pts',(-18.2968551847896,-16.8806071889227,
-18.317551744146));
#68758=CARTESIAN_POINT('Ctrl Pts',(-18.3053191833905,-16.8788390031324,
-18.3170358364379));
#68759=CARTESIAN_POINT('Ctrl Pts',(-18.3181721130978,-16.8762360138858,
-18.3162489893915));
#68760=CARTESIAN_POINT('Ctrl Pts',(-18.3225533635816,-16.8753631463077,
-18.3159801711957));
#68761=CARTESIAN_POINT('Ctrl Pts',(-18.3304337895588,-16.873819062592,-18.3154955225473));
#68762=CARTESIAN_POINT('Ctrl Pts',(-18.3339319222591,-16.8731428072905,
-18.315279982826));
#68763=CARTESIAN_POINT('Ctrl Pts',(-18.3415497639809,-16.8716900743654,
-18.3148097157304));
#68764=CARTESIAN_POINT('Ctrl Pts',(-18.3456700244796,-16.870917011781,-18.3145548026325));
#68765=CARTESIAN_POINT('Ctrl Pts',(-18.3572834573702,-16.8687737348109,
-18.3138347771251));
#68766=CARTESIAN_POINT('Ctrl Pts',(-18.3647816792995,-16.867431734609,-18.3133681076938));
#68767=CARTESIAN_POINT('Ctrl Pts',(-18.4094321068722,-16.8596888509005,
-18.3105792426965));
#68768=CARTESIAN_POINT('Ctrl Pts',(-18.4467402320654,-16.8542412717936,
-18.3082081649991));
#68769=CARTESIAN_POINT('Ctrl Pts',(-18.5704103869233,-16.8395441557004,
-18.3002571137243));
#68770=CARTESIAN_POINT('Ctrl Pts',(-18.6571933006942,-16.8346124412187,
-18.2945346038622));
#68771=CARTESIAN_POINT('Ctrl Pts',(-18.9147598837674,-16.8358324561702,
-18.2775169135569));
#68772=CARTESIAN_POINT('Ctrl Pts',(-19.084801403749,-16.857292691771,-18.2662989567347));
#68773=CARTESIAN_POINT('Ctrl Pts',(-19.2762097564064,-16.9054409816596,
-18.2541083349811));
#68774=CARTESIAN_POINT('Ctrl Pts',(-19.3018584799974,-16.9124088441307,
-18.2524823509199));
#68775=CARTESIAN_POINT('Ctrl Pts',(-19.3370961451349,-16.9226979772032,
-18.2502580194705));
#68776=CARTESIAN_POINT('Ctrl Pts',(-19.3468017509425,-16.9256077182263,
-18.2496463689467));
#68777=CARTESIAN_POINT('Ctrl Pts',(-19.3622940292873,-16.9303737893198,
-18.2486715527861));
#68778=CARTESIAN_POINT('Ctrl Pts',(-19.36809415871,-16.9321855228674,-18.2483069334462));
#68779=CARTESIAN_POINT('Ctrl Pts',(-19.3800345708687,-16.9359717429511,
-18.2475569834793));
#68780=CARTESIAN_POINT('Ctrl Pts',(-19.3861737973517,-16.937949370188,-18.2471717605544));
#68781=CARTESIAN_POINT('Ctrl Pts',(-19.4004378523211,-16.942616305479,-18.2462775337754));
#68782=CARTESIAN_POINT('Ctrl Pts',(-19.4085556385679,-16.9453268984285,
-18.2457692371758));
#68783=CARTESIAN_POINT('Ctrl Pts',(-19.4330556420134,-16.9536731153638,
-18.2442368731848));
#68784=CARTESIAN_POINT('Ctrl Pts',(-19.4493855825662,-16.9594607599333,
-18.2432178346807));
#68785=CARTESIAN_POINT('Ctrl Pts',(-19.4876382795282,-16.9735491517817,
-18.2408350647805));
#68786=CARTESIAN_POINT('Ctrl Pts',(-19.5094980762103,-16.9820149212567,
-18.2394767974568));
#68787=CARTESIAN_POINT('Ctrl Pts',(-19.5843781190441,-17.0124537643067,
-18.2348305730171));
#68788=CARTESIAN_POINT('Ctrl Pts',(-19.6366445080963,-17.0362191793076,
-18.2315996158654));
#68789=CARTESIAN_POINT('Ctrl Pts',(-19.7978121302769,-17.1175640011375,
-18.2215795037399));
#68790=CARTESIAN_POINT('Ctrl Pts',(-19.9026884797029,-17.1825314089948,
-18.2149861629799));
#68791=CARTESIAN_POINT('Ctrl Pts',(-20.0821187421126,-17.3166288804899,
-18.2027317641182));
#68792=CARTESIAN_POINT('Ctrl Pts',(-20.1584847322518,-17.3827005773451,
-18.1971273731389));
#68793=CARTESIAN_POINT('Ctrl Pts',(-20.2367001191189,-17.4608007143964,
-18.1905789943473));
#68794=CARTESIAN_POINT('Ctrl Pts',(-20.2435120032152,-17.4676966410243,
-18.190001369143));
#68795=CARTESIAN_POINT('Ctrl Pts',(-20.2534996574553,-17.4779473795998,
-18.1891431228434));
#68796=CARTESIAN_POINT('Ctrl Pts',(-20.2567122996807,-17.481266309562,-18.1888653037972));
#68797=CARTESIAN_POINT('Ctrl Pts',(-20.26239251635,-17.4871730131163,-18.1883709157996));
#68798=CARTESIAN_POINT('Ctrl Pts',(-20.2648644238387,-17.4897565520224,
-18.1881546887043));
#68799=CARTESIAN_POINT('Ctrl Pts',(-20.2701466396751,-17.4953053883241,
-18.1876902956425));
#68800=CARTESIAN_POINT('Ctrl Pts',(-20.2729548709297,-17.4982725169895,
-18.1874419833355));
#68801=CARTESIAN_POINT('Ctrl Pts',(-20.2787001087953,-17.5043781397853,
-18.1869310788197));
#68802=CARTESIAN_POINT('Ctrl Pts',(-20.2816361788512,-17.5075174859291,
-18.1866684185065));
#68803=CARTESIAN_POINT('Ctrl Pts',(-20.2950866022405,-17.5219872201699,
-18.1854580198056));
#68804=CARTESIAN_POINT('Ctrl Pts',(-20.3054859071369,-17.5334232689213,
-18.184502075058));
#68805=CARTESIAN_POINT('Ctrl Pts',(-20.3737946210223,-17.6102148361597,
-18.1780936618964));
#68806=CARTESIAN_POINT('Ctrl Pts',(-20.4277326240544,-17.6789797776092,
-18.1724087601117));
#68807=CARTESIAN_POINT('Ctrl Pts',(-20.5185471941585,-17.8107839014612,
-18.1618727497343));
#68808=CARTESIAN_POINT('Ctrl Pts',(-20.5567126316442,-17.8727865441772,
-18.1570468443867));
#68809=CARTESIAN_POINT('Ctrl Pts',(-20.5938784842887,-17.9407812358528,
-18.1519508018364));
#68810=CARTESIAN_POINT('Ctrl Pts',(-20.596132823833,-17.9449385758964,-18.1516399652404));
#68811=CARTESIAN_POINT('Ctrl Pts',(-20.6621274724152,-18.0676218725202,
-18.1424894559388));
#68812=CARTESIAN_POINT('Ctrl Pts',(-20.7144446144191,-18.1919664245569,
-18.1338570828094));
#68813=CARTESIAN_POINT('Ctrl Pts',(-20.7593064019422,-18.3355007146892,
-18.1246738597621));
#68814=CARTESIAN_POINT('Ctrl Pts',(-20.7638400038434,-18.350595834386,-18.1237169480434));
#68815=CARTESIAN_POINT('Ctrl Pts',(-20.7704400293477,-18.3734966198158,
-18.1222782877187));
#68816=CARTESIAN_POINT('Ctrl Pts',(-20.7726309949981,-18.3812655406726,
-18.1217924912484));
#68817=CARTESIAN_POINT('Ctrl Pts',(-20.7764755741626,-18.3952026350265,
-18.1209249741425));
#68818=CARTESIAN_POINT('Ctrl Pts',(-20.778145804565,-18.4013660855376,-18.1205427172853));
#68819=CARTESIAN_POINT('Ctrl Pts',(-20.7816287326791,-18.4144529871121,
-18.1197339702438));
#68820=CARTESIAN_POINT('Ctrl Pts',(-20.7834342647165,-18.4213782755158,
-18.1193077164557));
#68821=CARTESIAN_POINT('Ctrl Pts',(-20.7870376484727,-18.4354921883167,
-18.1184424317947));
#68822=CARTESIAN_POINT('Ctrl Pts',(-20.7888329462385,-18.4426813661912,
-18.1180034881602));
#68823=CARTESIAN_POINT('Ctrl Pts',(-20.7932123904979,-18.4606187545168,
-18.116912704427));
#68824=CARTESIAN_POINT('Ctrl Pts',(-20.7957501857015,-18.4713781359163,
-18.1162623491113));
#68825=CARTESIAN_POINT('Ctrl Pts',(-20.8334344639406,-18.6369398937002,
-18.1063131487805));
#68826=CARTESIAN_POINT('Ctrl Pts',(-20.8511450347541,-18.7951910216362,
-18.0976370133688));
#68827=CARTESIAN_POINT('Ctrl Pts',(-20.8509991056242,-18.9539459667055,
-18.0890147524363));
#68828=CARTESIAN_POINT('Ctrl Pts',(-20.850999105731,-18.9539458505088,-18.0890147587472));
#68829=CARTESIAN_POINT('Ctrl Pts',(-20.8508677551986,-19.096849407723,-18.0812534146201));
#68830=CARTESIAN_POINT('Ctrl Pts',(-20.8362671717255,-19.2393578459244,
-18.0735575723068));
#68831=CARTESIAN_POINT('Ctrl Pts',(-20.8054602106998,-19.3888487512122,
-18.0645864802766));
#68832=CARTESIAN_POINT('Ctrl Pts',(-20.8034244703069,-19.3983928649445,
-18.0640096594921));
#68833=CARTESIAN_POINT('Ctrl Pts',(-20.8001174997201,-19.4133879088025,
-18.0630965012489));
#68834=CARTESIAN_POINT('Ctrl Pts',(-20.798890487582,-19.4188485811966,-18.0627625166399));
#68835=CARTESIAN_POINT('Ctrl Pts',(-20.7965251623351,-19.4291834111655,
-18.0621275712305));
#68836=CARTESIAN_POINT('Ctrl Pts',(-20.7953911859381,-19.4340585343316,
-18.0618268523904));
#68837=CARTESIAN_POINT('Ctrl Pts',(-20.7934048894696,-19.4424627223062,
-18.0613062949401));
#68838=CARTESIAN_POINT('Ctrl Pts',(-20.7925607517554,-19.4459937367306,
-18.0610869260083));
#68839=CARTESIAN_POINT('Ctrl Pts',(-20.7909045652851,-19.4528435715514,
-18.0606600682991));
#68840=CARTESIAN_POINT('Ctrl Pts',(-20.7900935636639,-19.4561626036618,
-18.0604526460464));
#68841=CARTESIAN_POINT('Ctrl Pts',(-20.7878796790763,-19.465128757864,-18.0598907349418));
#68842=CARTESIAN_POINT('Ctrl Pts',(-20.7864615546186,-19.470772033985,-18.0595353804882));
#68843=CARTESIAN_POINT('Ctrl Pts',(-20.7810870793073,-19.4917921744127,
-18.0582056344514));
#68844=CARTESIAN_POINT('Ctrl Pts',(-20.7769811537,-19.5071297803452,-18.0572231410393));
#68845=CARTESIAN_POINT('Ctrl Pts',(-20.7579998303821,-19.5749698604786,
-18.052827473929));
#68846=CARTESIAN_POINT('Ctrl Pts',(-20.7412777861463,-19.626904783481,-18.049329319184));
#68847=CARTESIAN_POINT('Ctrl Pts',(-20.7225806448396,-19.6781101975385,
-18.0457833736847));
#68848=CARTESIAN_POINT('Origin',(-18.734,-18.952,0.));
#68849=CARTESIAN_POINT('',(-20.7225805822089,-19.6781103690637,-17.242699000807));
#68850=CARTESIAN_POINT('',(-20.7225805818549,-19.6781103700332,-17.4677765722177));
#68851=CARTESIAN_POINT('',(-20.7225805821191,-19.6781103693095,0.));
#68852=CARTESIAN_POINT('Ctrl Pts',(-20.7225805818549,-19.6781103700332,
-17.4677765722177));
#68853=CARTESIAN_POINT('Ctrl Pts',(-20.7401854861152,-19.6298962524523,
-17.471069514147));
#68854=CARTESIAN_POINT('Ctrl Pts',(-20.7560325913588,-19.5810537941813,
-17.474316044063));
#68855=CARTESIAN_POINT('Ctrl Pts',(-20.7795153229111,-19.4985720222208,
-17.4796471969592));
#68856=CARTESIAN_POINT('Ctrl Pts',(-20.7881324598313,-19.4652387044823,
-17.4817615361231));
#68857=CARTESIAN_POINT('Ctrl Pts',(-20.7983855430847,-19.4211678249985,
-17.4845062026776));
#68858=CARTESIAN_POINT('Ctrl Pts',(-20.8007569917464,-19.4106083976442,
-17.4851600453581));
#68859=CARTESIAN_POINT('Ctrl Pts',(-20.8045078951291,-19.3932863925522,
-17.4862265621788));
#68860=CARTESIAN_POINT('Ctrl Pts',(-20.8059354161732,-19.3865345291287,
-17.4866407714016));
#68861=CARTESIAN_POINT('Ctrl Pts',(-20.8086343585082,-19.3734533809918,
-17.4874404011248));
#68862=CARTESIAN_POINT('Ctrl Pts',(-20.8099098928274,-19.3671250319341,
-17.4878259492365));
#68863=CARTESIAN_POINT('Ctrl Pts',(-20.8127876275962,-19.3525026283939,
-17.4887138658021));
#68864=CARTESIAN_POINT('Ctrl Pts',(-20.8143691793209,-19.3442045854958,
-17.4892155706158));
#68865=CARTESIAN_POINT('Ctrl Pts',(-20.8184877290584,-19.321869406054,-17.4905602545672));
#68866=CARTESIAN_POINT('Ctrl Pts',(-20.8209326204345,-19.3078155740382,
-17.4914003056032));
#68867=CARTESIAN_POINT('Ctrl Pts',(-20.8418093117342,-19.1801846375292,
-17.4989769688998));
#68868=CARTESIAN_POINT('Ctrl Pts',(-20.8510962905051,-19.0652992221111,
-17.5054071708765));
#68869=CARTESIAN_POINT('Ctrl Pts',(-20.8508421940714,-18.7639639427916,
-17.5219135939307));
#68870=CARTESIAN_POINT('Ctrl Pts',(-20.8261075481732,-18.5785810131941,
-17.5316811786551));
#68871=CARTESIAN_POINT('Ctrl Pts',(-20.7737437540389,-18.3851344241272,
-17.5434581358864));
#68872=CARTESIAN_POINT('Ctrl Pts',(-20.7698906309289,-18.3714481266278,
-17.5443005254895));
#68873=CARTESIAN_POINT('Ctrl Pts',(-20.7643392700289,-18.3524648712353,
-17.5454830647105));
#68874=CARTESIAN_POINT('Ctrl Pts',(-20.7627574775413,-18.3471338844243,
-17.5458167097691));
#68875=CARTESIAN_POINT('Ctrl Pts',(-20.7601843572634,-18.3385855526011,
-17.5463543107302));
#68876=CARTESIAN_POINT('Ctrl Pts',(-20.7592063133516,-18.33536419023,-17.5465574940822));
#68877=CARTESIAN_POINT('Ctrl Pts',(-20.757146922833,-18.3286389689199,-17.5469829456692));
#68878=CARTESIAN_POINT('Ctrl Pts',(-20.7560641559174,-18.3251355847886,
-17.5472052993924));
#68879=CARTESIAN_POINT('Ctrl Pts',(-20.7534222731797,-18.3166656150336,
-17.5477445943649));
#68880=CARTESIAN_POINT('Ctrl Pts',(-20.7518539351081,-18.3117019495744,
-17.5480620717639));
#68881=CARTESIAN_POINT('Ctrl Pts',(-20.7463005713028,-18.2943490398617,
-17.5491768673399));
#68882=CARTESIAN_POINT('Ctrl Pts',(-20.7422197140405,-18.2819910930458,
-17.5499795316202));
#68883=CARTESIAN_POINT('Ctrl Pts',(-20.7174287695851,-18.2091790822462,
-17.5547574141077));
#68884=CARTESIAN_POINT('Ctrl Pts',(-20.694105627527,-18.1496553270635,-17.5588616249813));
#68885=CARTESIAN_POINT('Ctrl Pts',(-20.5919079167676,-17.920005290123,-17.5752529078129));
#68886=CARTESIAN_POINT('Ctrl Pts',(-20.4932542179064,-17.7595743407234,
-17.5878515668483));
#68887=CARTESIAN_POINT('Ctrl Pts',(-20.3393459548716,-17.5708073277645,
-17.6032549052734));
#68888=CARTESIAN_POINT('Ctrl Pts',(-20.3022245158644,-17.5287988102026,
-17.6067354644614));
#68889=CARTESIAN_POINT('Ctrl Pts',(-20.255157559347,-17.4796164013013,-17.6108793950905));
#68890=CARTESIAN_POINT('Ctrl Pts',(-20.2467641838835,-17.4709941541593,
-17.6116086314705));
#68891=CARTESIAN_POINT('Ctrl Pts',(-20.2327633598476,-17.456854770822,-17.6128092320561));
#68892=CARTESIAN_POINT('Ctrl Pts',(-20.2271979436423,-17.4512965753145,
-17.61328242557));
#68893=CARTESIAN_POINT('Ctrl Pts',(-20.2170712612416,-17.4412951387361,
-17.6141361980115));
#68894=CARTESIAN_POINT('Ctrl Pts',(-20.2125207008507,-17.4368412352841,
-17.6145172454367));
#68895=CARTESIAN_POINT('Ctrl Pts',(-20.202714665704,-17.4273297313886,-17.6153328385272));
#68896=CARTESIAN_POINT('Ctrl Pts',(-20.197452997426,-17.4222786124235,-17.615767098652));
#68897=CARTESIAN_POINT('Ctrl Pts',(-20.1830323070875,-17.4085774787785,
-17.6169482259019));
#68898=CARTESIAN_POINT('Ctrl Pts',(-20.1738219181304,-17.3999817783296,
-17.6176927481422));
#68899=CARTESIAN_POINT('Ctrl Pts',(-20.1246868229696,-17.3549397587563,
-17.6216138226633));
#68900=CARTESIAN_POINT('Ctrl Pts',(-20.0834517989649,-17.3199485854839,
-17.624728530735));
#68901=CARTESIAN_POINT('Ctrl Pts',(-19.8904575622519,-17.1684992483461,
-17.6386248336708));
#68902=CARTESIAN_POINT('Ctrl Pts',(-19.7247043987413,-17.0713702819603,
-17.6486489049994));
#68903=CARTESIAN_POINT('Ctrl Pts',(-19.5328954563912,-16.9914570081762,
-17.6601999008382));
#68904=CARTESIAN_POINT('Ctrl Pts',(-19.5175481405615,-16.9852730071484,
-17.6611244838335));
#68905=CARTESIAN_POINT('Ctrl Pts',(-19.4525654555233,-16.9599704292826,
-17.6650467943258));
#68906=CARTESIAN_POINT('Ctrl Pts',(-19.4022953006937,-16.9425477103398,
-17.668099220139));
#68907=CARTESIAN_POINT('Ctrl Pts',(-19.3430953509111,-16.9244971691108,
-17.6717720662578));
#68908=CARTESIAN_POINT('Ctrl Pts',(-19.3347479435923,-16.9220081827417,
-17.6722917359694));
#68909=CARTESIAN_POINT('Ctrl Pts',(-19.3220834208956,-16.9183168951466,
-17.6730831997672));
#68910=CARTESIAN_POINT('Ctrl Pts',(-19.3177773400454,-16.9170766360133,
-17.6733528351883));
#68911=CARTESIAN_POINT('Ctrl Pts',(-19.3100396639071,-16.9148745726947,
-17.6738383501984));
#68912=CARTESIAN_POINT('Ctrl Pts',(-19.3066095517231,-16.9139077543091,
-17.6740539343943));
#68913=CARTESIAN_POINT('Ctrl Pts',(-19.2991494813891,-16.911825363292,-17.6745235868459));
#68914=CARTESIAN_POINT('Ctrl Pts',(-19.295118707193,-16.9107130823128,-17.6747778369294));
#68915=CARTESIAN_POINT('Ctrl Pts',(-19.2837834659244,-16.9076212643585,
-17.6754941578965));
#68916=CARTESIAN_POINT('Ctrl Pts',(-19.2764717266792,-16.9056689671687,
-17.6759577608106));
#68917=CARTESIAN_POINT('Ctrl Pts',(-19.2326183085346,-16.8942112758065,
-17.6787468758586));
#68918=CARTESIAN_POINT('Ctrl Pts',(-19.1958405304369,-16.8856463111251,
-17.6811214910051));
#68919=CARTESIAN_POINT('Ctrl Pts',(-19.0738764096172,-16.8606612779821,
-17.68906959481));
#68920=CARTESIAN_POINT('Ctrl Pts',(-18.9879122289604,-16.8484933339368,
-17.6947851606618));
#68921=CARTESIAN_POINT('Ctrl Pts',(-18.7261823111601,-16.8277259621054,
-17.7121319592443));
#68922=CARTESIAN_POINT('Ctrl Pts',(-18.5498275851324,-16.835704789497,-17.7236766568872));
#68923=CARTESIAN_POINT('Ctrl Pts',(-18.3538340284923,-16.8692877840743,
-17.7359159094666));
#68924=CARTESIAN_POINT('Ctrl Pts',(-18.3312639400846,-16.8735342024731,
-17.7373177514194));
#68925=CARTESIAN_POINT('Ctrl Pts',(-18.2994195019062,-16.8800637476046,
-17.7392855358154));
#68926=CARTESIAN_POINT('Ctrl Pts',(-18.2900852584993,-16.8820435390437,
-17.7398611017316));
#68927=CARTESIAN_POINT('Ctrl Pts',(-18.2749369402658,-16.8853636748998,
-17.740793252841));
#68928=CARTESIAN_POINT('Ctrl Pts',(-18.2691146619857,-16.8866655920486,
-17.7411510639488));
#68929=CARTESIAN_POINT('Ctrl Pts',(-18.2569360423183,-16.8894429562582,
-17.7418985679055));
#68930=CARTESIAN_POINT('Ctrl Pts',(-18.2505808540461,-16.8909232160826,
-17.74228810183));
#68931=CARTESIAN_POINT('Ctrl Pts',(-18.2354732429854,-16.894515823417,-17.7432128746599));
#68932=CARTESIAN_POINT('Ctrl Pts',(-18.2267272065016,-16.8966546808044,
-17.7437472544271));
#68933=CARTESIAN_POINT('Ctrl Pts',(-18.197284262263,-16.9040543846259,-17.7455430827491));
#68934=CARTESIAN_POINT('Ctrl Pts',(-18.176652961178,-16.909572680828,-17.7467962201684));
#68935=CARTESIAN_POINT('Ctrl Pts',(-18.0646398377423,-16.9413568062523,
-17.7535764826653));
#68936=CARTESIAN_POINT('Ctrl Pts',(-17.975018359019,-16.9734452245979,-17.7589092896504));
#68937=CARTESIAN_POINT('Ctrl Pts',(-17.7316741726181,-17.0795524129059,
-17.7735143763218));
#68938=CARTESIAN_POINT('Ctrl Pts',(-17.5843097503121,-17.1662459757609,
-17.7824772334188));
#68939=CARTESIAN_POINT('Ctrl Pts',(-17.4194318623883,-17.2921871970481,
-17.7943233017074));
#68940=CARTESIAN_POINT('Ctrl Pts',(-17.3905221604003,-17.3154992064986,
-17.7964797261972));
#68941=CARTESIAN_POINT('Ctrl Pts',(-17.3567866104648,-17.3441991451115,
-17.799112841559));
#68942=CARTESIAN_POINT('Ctrl Pts',(-17.3513544538886,-17.348868190131,-17.7995405541146));
#68943=CARTESIAN_POINT('Ctrl Pts',(-17.3425342763275,-17.3565274808376,
-17.8002413280508));
#68944=CARTESIAN_POINT('Ctrl Pts',(-17.3391318992228,-17.3595012087532,
-17.8005131948968));
#68945=CARTESIAN_POINT('Ctrl Pts',(-17.3330612455963,-17.3648414299601,
-17.8010010950864));
#68946=CARTESIAN_POINT('Ctrl Pts',(-17.3303894056283,-17.3672037925531,
-17.8012168203345));
#68947=CARTESIAN_POINT('Ctrl Pts',(-17.3246189958244,-17.3723318592769,
-17.8016848832848));
#68948=CARTESIAN_POINT('Ctrl Pts',(-17.3215226340736,-17.3750998954252,
-17.8019373925274));
#68949=CARTESIAN_POINT('Ctrl Pts',(-17.3129034377732,-17.3828509016506,
-17.8026440171153));
#68950=CARTESIAN_POINT('Ctrl Pts',(-17.3073987545363,-17.3878538384509,
-17.8030995999471));
#68951=CARTESIAN_POINT('Ctrl Pts',(-17.2757195551927,-17.4169518489541,
-17.8057458069974));
#68952=CARTESIAN_POINT('Ctrl Pts',(-17.25013101886,-17.4416731536205,-17.8079799766362));
#68953=CARTESIAN_POINT('Ctrl Pts',(-17.170135650724,-17.5229531200549,-17.8152468071432));
#68954=CARTESIAN_POINT('Ctrl Pts',(-17.118247789956,-17.5818942296853,-17.8203977703006));
#68955=CARTESIAN_POINT('Ctrl Pts',(-16.953492832108,-17.7914534657815,-17.8379924651614));
#68956=CARTESIAN_POINT('Ctrl Pts',(-16.8574322263416,-17.9542043349617,
-17.850398086955));
#68957=CARTESIAN_POINT('Ctrl Pts',(-16.7756371588606,-18.1476487008244,
-17.8633108495524));
#68958=CARTESIAN_POINT('Ctrl Pts',(-16.7674427358968,-18.167896299497,-17.8646431667679));
#68959=CARTESIAN_POINT('Ctrl Pts',(-16.756526405379,-18.1961177171648,-17.866474275795));
#68960=CARTESIAN_POINT('Ctrl Pts',(-16.7535367473027,-18.2039858618691,
-17.8669820337858));
#68961=CARTESIAN_POINT('Ctrl Pts',(-16.7484730049532,-18.2175557481883,
-17.8678530725593));
#68962=CARTESIAN_POINT('Ctrl Pts',(-16.7463763772549,-18.2232489159007,
-17.8682171046256));
#68963=CARTESIAN_POINT('Ctrl Pts',(-16.7420995917008,-18.235017831786,-17.8689667624978));
#68964=CARTESIAN_POINT('Ctrl Pts',(-16.7399226884386,-18.2410947017641,
-17.8693522765633));
#68965=CARTESIAN_POINT('Ctrl Pts',(-16.7349133460213,-18.2552824414518,
-17.8702487306718));
#68966=CARTESIAN_POINT('Ctrl Pts',(-16.7321024046534,-18.263400822271,-17.8707589524153));
#68967=CARTESIAN_POINT('Ctrl Pts',(-16.7232311904579,-18.289535584376,-17.8723928486743));
#68968=CARTESIAN_POINT('Ctrl Pts',(-16.7173640073555,-18.3076168721773,
-17.8735101488881));
#68969=CARTESIAN_POINT('Ctrl Pts',(-16.6891047480586,-18.3988741001927,
-17.8790869964669));
#68970=CARTESIAN_POINT('Ctrl Pts',(-16.6704471663584,-18.4731510172963,
-17.8834235159508));
#68971=CARTESIAN_POINT('Ctrl Pts',(-16.6348971005142,-18.6561457115751,
-17.8937835424958));
#68972=CARTESIAN_POINT('Ctrl Pts',(-16.6223719831967,-18.7654773956982,
-17.8996976506881));
#68973=CARTESIAN_POINT('Ctrl Pts',(-16.6158517440397,-18.9453001108026,
-17.9094975582051));
#68974=CARTESIAN_POINT('Ctrl Pts',(-16.6167901534409,-19.0153896009238,
-17.9133382942622));
#68975=CARTESIAN_POINT('Ctrl Pts',(-16.6226174751437,-19.1077530992226,
-17.9185657552509));
#68976=CARTESIAN_POINT('Ctrl Pts',(-16.6243919466964,-19.1301824547245,
-17.9198482894585));
#68977=CARTESIAN_POINT('Ctrl Pts',(-16.6291864459383,-19.180558218768,-17.9227666829439));
#68978=CARTESIAN_POINT('Ctrl Pts',(-16.6324062069207,-19.208480629486,-17.9244106055936));
#68979=CARTESIAN_POINT('Ctrl Pts',(-16.6371419761922,-19.2434217874193,
-17.9265100428424));
#68980=CARTESIAN_POINT('Ctrl Pts',(-16.6381392346461,-19.250509428852,-17.9269380957575));
#68981=CARTESIAN_POINT('Ctrl Pts',(-16.6397691328093,-19.2616823598337,
-17.9276165300285));
#68982=CARTESIAN_POINT('Ctrl Pts',(-16.6403778405237,-19.2657711614613,
-17.9278655802577));
#68983=CARTESIAN_POINT('Ctrl Pts',(-16.6415343445789,-19.2733863979493,
-17.9283309116397));
#68984=CARTESIAN_POINT('Ctrl Pts',(-16.6420790832379,-19.2769132396271,
-17.9285470184905));
#68985=CARTESIAN_POINT('Ctrl Pts',(-16.6433380160572,-19.2849296245236,
-17.9290395748299));
#68986=CARTESIAN_POINT('Ctrl Pts',(-16.644057752191,-19.289418235905,-17.9293163340189));
#68987=CARTESIAN_POINT('Ctrl Pts',(-16.6462971863751,-19.3031023047266,
-17.9301629313079));
#68988=CARTESIAN_POINT('Ctrl Pts',(-16.6478631337355,-19.3122899308938,
-17.9307352940335));
#68989=CARTESIAN_POINT('Ctrl Pts',(-16.6690630663666,-19.4318987510933,
-17.9382354395378));
#68990=CARTESIAN_POINT('Ctrl Pts',(-16.697378932201,-19.5405881364994,-17.9455856423567));
#68991=CARTESIAN_POINT('Ctrl Pts',(-16.7954140475729,-19.822879879384,-17.9653126596922));
#68992=CARTESIAN_POINT('Ctrl Pts',(-16.8797423009026,-19.9904140676861,
-17.9776195768835));
#68993=CARTESIAN_POINT('Ctrl Pts',(-16.9973638158794,-20.1628952612935,
-17.9904569702309));
#68994=CARTESIAN_POINT('Ctrl Pts',(-17.0100358787283,-20.1808695356474,
-17.9917985229709));
#68995=CARTESIAN_POINT('Ctrl Pts',(-17.0279565165576,-20.205465546407,-17.9936401846737));
#68996=CARTESIAN_POINT('Ctrl Pts',(-17.0329677550768,-20.2122577309365,
-17.9941493950113));
#68997=CARTESIAN_POINT('Ctrl Pts',(-17.0416542973813,-20.2238851779148,
-17.9950222637246));
#68998=CARTESIAN_POINT('Ctrl Pts',(-17.0453100037779,-20.2287348905807,
-17.9953866805701));
#68999=CARTESIAN_POINT('Ctrl Pts',(-17.052892133641,-20.238703914709,-17.9961365283828));
#69000=CARTESIAN_POINT('Ctrl Pts',(-17.0568211945744,-20.2438211480367,
-17.9965218502619));
#69001=CARTESIAN_POINT('Ctrl Pts',(-17.066023445091,-20.2556934637922,-17.997416837854));
#69002=CARTESIAN_POINT('Ctrl Pts',(-17.0713144040846,-20.26243467891,-17.9979257925395));
#69003=CARTESIAN_POINT('Ctrl Pts',(-17.0883990241637,-20.283932151617,-17.9995514806227));
#69004=CARTESIAN_POINT('Ctrl Pts',(-17.1003495162504,-20.2985630172221,
-18.0006619306715));
#69005=CARTESIAN_POINT('Ctrl Pts',(-17.1611267347661,-20.3709717249482,
-18.0061812600895));
#69006=CARTESIAN_POINT('Ctrl Pts',(-17.2128322848691,-20.4262664574954,
-18.0104700605032));
#69007=CARTESIAN_POINT('Ctrl Pts',(-17.3462271448384,-20.5544125889058,
-18.0207555885344));
#69008=CARTESIAN_POINT('Ctrl Pts',(-17.4308125953392,-20.6239279523162,
-18.026642361794));
#69009=CARTESIAN_POINT('Ctrl Pts',(-17.6175210890745,-20.7545584837677,
-18.0390483178221));
#69010=CARTESIAN_POINT('Ctrl Pts',(-17.7201773575577,-20.8142292450865,
-18.0455602415365));
#69011=CARTESIAN_POINT('Ctrl Pts',(-17.8358751192896,-20.869068441837,-18.0531480800421));
#69012=CARTESIAN_POINT('Ctrl Pts',(-17.8445088197518,-20.8730895722569,
-18.0537157704433));
#69013=CARTESIAN_POINT('Ctrl Pts',(-17.8573395695598,-20.8789604363245,
-18.0545620164123));
#69014=CARTESIAN_POINT('Ctrl Pts',(-17.8615161076739,-20.8808550723636,
-18.0548378817539));
#69015=CARTESIAN_POINT('Ctrl Pts',(-17.8689567843353,-20.8842013344618,
-18.0553301216175));
#69016=CARTESIAN_POINT('Ctrl Pts',(-17.8722184733929,-20.8856582847119,
-18.0555461653519));
#69017=CARTESIAN_POINT('Ctrl Pts',(-17.87923762588,-20.8887723531228,-18.0560116782155));
#69018=CARTESIAN_POINT('Ctrl Pts',(-17.8829961725166,-20.8904267716317,
-18.0562613016241));
#69019=CARTESIAN_POINT('Ctrl Pts',(-17.8933810528223,-20.8949619123441,
-18.0569519423051));
#69020=CARTESIAN_POINT('Ctrl Pts',(-17.9000172851446,-20.8978196306515,
-18.0573943233906));
#69021=CARTESIAN_POINT('Ctrl Pts',(-17.936401001052,-20.913267001808,-18.0598248828219));
#69022=CARTESIAN_POINT('Ctrl Pts',(-17.9664173000941,-20.9252077819085,
-18.061848872269));
#69023=CARTESIAN_POINT('Ctrl Pts',(-18.149395863999,-20.9931918247272,-18.0742498508666));
#69024=CARTESIAN_POINT('Ctrl Pts',(-18.308132352176,-21.032111224602,-18.0852205525414));
#69025=CARTESIAN_POINT('Ctrl Pts',(-18.5857202943358,-21.0670323183666,
-18.1034957546379));
#69026=CARTESIAN_POINT('Ctrl Pts',(-18.7027036719987,-21.0719945605717,
-18.1109407661892));
#69027=CARTESIAN_POINT('Ctrl Pts',(-18.8337944032507,-21.0666948446787,
-18.1189517061858));
#69028=CARTESIAN_POINT('Ctrl Pts',(-18.8480669670608,-21.065973025319,-18.1198197331435));
#69029=CARTESIAN_POINT('Ctrl Pts',(-18.8707706118965,-21.0645942067892,
-18.1211941068338));
#69030=CARTESIAN_POINT('Ctrl Pts',(-18.8792067632627,-21.0640311271334,
-18.1217033820663));
#69031=CARTESIAN_POINT('Ctrl Pts',(-18.8940791427192,-21.0629489235369,
-18.122598777195));
#69032=CARTESIAN_POINT('Ctrl Pts',(-18.9005167507343,-21.0624508672018,
-18.1229855532969));
#69033=CARTESIAN_POINT('Ctrl Pts',(-18.9138269366389,-21.0613598210612,
-18.1237836187335));
#69034=CARTESIAN_POINT('Ctrl Pts',(-18.9206991042232,-21.0607626770365,
-18.1241947727285));
#69035=CARTESIAN_POINT('Ctrl Pts',(-18.9383312239533,-21.059143698998,-18.1252474505101));
#69036=CARTESIAN_POINT('Ctrl Pts',(-18.9490865755848,-21.0580730255312,
-18.1258874331789));
#69037=CARTESIAN_POINT('Ctrl Pts',(-18.9939389302393,-21.0532608901094,
-18.128547844724));
#69038=CARTESIAN_POINT('Ctrl Pts',(-19.0279517884252,-21.0487732634634,
-18.1305447505903));
#69039=CARTESIAN_POINT('Ctrl Pts',(-19.1162738059897,-21.034928551885,-18.1356881264718));
#69040=CARTESIAN_POINT('Ctrl Pts',(-19.1703541838453,-21.0242741822414,
-18.1387952215826));
#69041=CARTESIAN_POINT('Ctrl Pts',(-19.3893465596709,-20.9721758682196,
-18.1513119061741));
#69042=CARTESIAN_POINT('Ctrl Pts',(-19.5493765534055,-20.9130568436342,
-18.1602560318618));
#69043=CARTESIAN_POINT('Ctrl Pts',(-19.7072213182256,-20.8320490854616,
-18.1701910795476));
#69044=CARTESIAN_POINT('Ctrl Pts',(-19.7138191888339,-20.8286189419307,
-18.17060861938));
#69045=CARTESIAN_POINT('Ctrl Pts',(-19.7661388625077,-20.801067518496,-18.1739386610872));
#69046=CARTESIAN_POINT('Ctrl Pts',(-19.8109774221947,-20.7753156653979,
-18.1769084506207));
#69047=CARTESIAN_POINT('Ctrl Pts',(-19.8621009869288,-20.7434102629205,
-18.1804851115094));
#69048=CARTESIAN_POINT('Ctrl Pts',(-19.869349551062,-20.7388251056207,-18.1809968357557));
#69049=CARTESIAN_POINT('Ctrl Pts',(-19.8802770325903,-20.7318194727903,
-18.1817755946933));
#69050=CARTESIAN_POINT('Ctrl Pts',(-19.8839766894152,-20.7294312937958,
-18.1820405339688));
#69051=CARTESIAN_POINT('Ctrl Pts',(-19.8905140982894,-20.7251823526583,
-18.1825110095978));
#69052=CARTESIAN_POINT('Ctrl Pts',(-19.8933548548627,-20.7233262928215,
-18.1827162308012));
#69053=CARTESIAN_POINT('Ctrl Pts',(-19.8962134283951,-20.7214487694101,
-18.1829235345918));
#69054=CARTESIAN_POINT('Ctrl Pts',(-19.8962356816485,-20.7214341527765,
-18.1829251484465));
#69055=CARTESIAN_POINT('Ctrl Pts',(-19.8962797191912,-20.7214052263504,
-18.1829283422414));
#69056=CARTESIAN_POINT('Ctrl Pts',(-19.8963015032605,-20.7213909167275,
-18.1829299221637));
#69057=CARTESIAN_POINT('Ctrl Pts',(-19.8963446318564,-20.7213625850703,
-18.1829330502217));
#69058=CARTESIAN_POINT('Ctrl Pts',(-19.8963659759384,-20.7213485633512,
-18.1829345983233));
#69059=CARTESIAN_POINT('Ctrl Pts',(-19.8964082500977,-20.7213207907929,
-18.1829376645868));
#69060=CARTESIAN_POINT('Ctrl Pts',(-19.8964291804592,-20.7213070397882,
-18.1829391827675));
#69061=CARTESIAN_POINT('Ctrl Pts',(-19.8964706525528,-20.7212797920503,
-18.1829421910247));
#69062=CARTESIAN_POINT('Ctrl Pts',(-19.8964911941522,-20.7212662954238,
-18.18294368109));
#69063=CARTESIAN_POINT('Ctrl Pts',(-19.8965319108553,-20.7212395419575,
-18.1829466347172));
#69064=CARTESIAN_POINT('Ctrl Pts',(-19.8965520863329,-20.72122628489,-18.1829480983047));
#69065=CARTESIAN_POINT('Ctrl Pts',(-19.8965920920005,-20.7211999966598,
-18.1829510005107));
#69066=CARTESIAN_POINT('Ctrl Pts',(-19.8966119224368,-20.7211869653519,
-18.1829524391455));
#69067=CARTESIAN_POINT('Ctrl Pts',(-19.8966512586304,-20.7211611151475,
-18.1829552929372));
#69068=CARTESIAN_POINT('Ctrl Pts',(-19.8966707640526,-20.7211482964868,
-18.1829567080684));
#69069=CARTESIAN_POINT('Ctrl Pts',(-19.8967094685502,-20.7211228595752,
-18.182959516179));
#69070=CARTESIAN_POINT('Ctrl Pts',(-19.896728667493,-20.7211102414258,-18.1829609091476));
#69071=CARTESIAN_POINT('Ctrl Pts',(-19.8967667755203,-20.7210851947428,
-18.1829636741259));
#69072=CARTESIAN_POINT('Ctrl Pts',(-19.8967856849602,-20.7210727659889,
-18.1829650461603));
#69073=CARTESIAN_POINT('Ctrl Pts',(-19.896823230357,-20.7210480873734,-18.1829677704551));
#69074=CARTESIAN_POINT('Ctrl Pts',(-19.8968418663888,-20.721035837475,-18.1829691227199));
#69075=CARTESIAN_POINT('Ctrl Pts',(-19.8968788806954,-20.7210115062702,
-18.1829718086137));
#69076=CARTESIAN_POINT('Ctrl Pts',(-19.8968972586385,-20.7209994251935,
-18.1829731422177));
#69077=CARTESIAN_POINT('Ctrl Pts',(-19.8969337709767,-20.7209754223258,
-18.1829757918182));
#69078=CARTESIAN_POINT('Ctrl Pts',(-19.896951905184,-20.7209635006692,-18.1829771078001));
#69079=CARTESIAN_POINT('Ctrl Pts',(-19.8969879426736,-20.7209398083753,
-18.1829797230699));
#69080=CARTESIAN_POINT('Ctrl Pts',(-19.8970058463033,-20.7209280375197,
-18.1829810223822));
#69081=CARTESIAN_POINT('Ctrl Pts',(-19.8970414351949,-20.720904638602,-18.1829836052215));
#69082=CARTESIAN_POINT('Ctrl Pts',(-19.8970591206562,-20.7208930104182,
-18.1829848887623));
#69083=CARTESIAN_POINT('Ctrl Pts',(-19.8970942864667,-20.7208698881563,
-18.1829874410185));
#69084=CARTESIAN_POINT('Ctrl Pts',(-19.8971117662386,-20.7208583944666,
-18.1829887096913));
#69085=CARTESIAN_POINT('Ctrl Pts',(-19.897146530569,-20.7208355347101,-18.1829912329278));
#69086=CARTESIAN_POINT('Ctrl Pts',(-19.8971638154642,-20.7208241684302,
-18.1829924875154));
#69087=CARTESIAN_POINT('Ctrl Pts',(-19.8971982013371,-20.7208015560897,
-18.1829949833993));
#69088=CARTESIAN_POINT('Ctrl Pts',(-19.8972153022018,-20.720790310111,-18.1829962246868));
#69089=CARTESIAN_POINT('Ctrl Pts',(-19.8972493300429,-20.7207679318003,
-18.182998694697));
#69090=CARTESIAN_POINT('Ctrl Pts',(-19.8972662569826,-20.7207567994996,
-18.1829999234163));
#69091=CARTESIAN_POINT('Ctrl Pts',(-19.8972999465503,-20.7207346422679,
-18.1830023689834));
#69092=CARTESIAN_POINT('Ctrl Pts',(-19.8973167091712,-20.7207236173483,
-18.1830035858302));
#69093=CARTESIAN_POINT('Ctrl Pts',(-19.8973500793006,-20.7207016688482,
-18.1830060083183));
#69094=CARTESIAN_POINT('Ctrl Pts',(-19.8973666868106,-20.720690745273,-18.1830072139593));
#69095=CARTESIAN_POINT('Ctrl Pts',(-19.8973997550678,-20.7206689939885,
-18.1830096146406));
#69096=CARTESIAN_POINT('Ctrl Pts',(-19.8974162160191,-20.7206581661508,
-18.1830108096952));
#69097=CARTESIAN_POINT('Ctrl Pts',(-19.8974489997398,-20.7206366007143,
-18.1830131898253));
#69098=CARTESIAN_POINT('Ctrl Pts',(-19.8974653224463,-20.7206258631623,
-18.1830143748958));
#69099=CARTESIAN_POINT('Ctrl Pts',(-19.8974978379949,-20.720604472842,-18.1830167356602));
#69100=CARTESIAN_POINT('Ctrl Pts',(-19.8975140305315,-20.7205938202798,
-18.1830179113315));
#69101=CARTESIAN_POINT('Ctrl Pts',(-19.9010411141942,-20.7182733931061,
-18.1832740034795));
#69102=CARTESIAN_POINT('Ctrl Pts',(-19.9045450846592,-20.7159531925442,
-18.1835296228759));
#69103=CARTESIAN_POINT('Ctrl Pts',(-19.9146520459037,-20.7092173582621,
-18.1842703754439));
#69104=CARTESIAN_POINT('Ctrl Pts',(-19.9212370382047,-20.7047750306903,
-18.1847572541746));
#69105=CARTESIAN_POINT('Ctrl Pts',(-19.9650511532819,-20.6748572402252,
-18.1880244528397));
#69106=CARTESIAN_POINT('Ctrl Pts',(-20.0014799916308,-20.6482363683382,
-18.1908749773723));
#69107=CARTESIAN_POINT('Ctrl Pts',(-20.1318630099769,-20.5464112232603,
-18.2014991280105));
#69108=CARTESIAN_POINT('Ctrl Pts',(-20.2202075162418,-20.4643999648833,
-18.2095229599269));
#69109=CARTESIAN_POINT('Ctrl Pts',(-20.3988404465469,-20.2677230962314,
-18.2270189211216));
#69110=CARTESIAN_POINT('Ctrl Pts',(-20.4852486801041,-20.150316983744,-18.236382428185));
#69111=CARTESIAN_POINT('Ctrl Pts',(-20.5661837883021,-20.0126579127701,
-18.2461327768856));
#69112=CARTESIAN_POINT('Ctrl Pts',(-20.5732919825117,-20.0002831968325,
-18.2469995817129));
#69113=CARTESIAN_POINT('Ctrl Pts',(-20.584408696955,-19.9804687840582,-18.248372392136));
#69114=CARTESIAN_POINT('Ctrl Pts',(-20.5884986450101,-19.9730754939952,
-18.2488813158762));
#69115=CARTESIAN_POINT('Ctrl Pts',(-20.5956354296389,-19.9599901808339,
-18.2497763022316));
#69116=CARTESIAN_POINT('Ctrl Pts',(-20.5987006749914,-19.954308371542,-18.2501630191671));
#69117=CARTESIAN_POINT('Ctrl Pts',(-20.604988339472,-19.9425247335344,-18.2509611630096));
#69118=CARTESIAN_POINT('Ctrl Pts',(-20.6082070156386,-19.9364209863916,
-18.2513724535886));
#69119=CARTESIAN_POINT('Ctrl Pts',(-20.6163954079357,-19.9207071674811,
-18.2524258964183));
#69120=CARTESIAN_POINT('Ctrl Pts',(-20.621321442429,-19.9110744640908,-18.2530665031507));
#69121=CARTESIAN_POINT('Ctrl Pts',(-20.6415981741794,-19.8706627081341,
-18.2557329865273));
#69122=CARTESIAN_POINT('Ctrl Pts',(-20.6562719922963,-19.8395486190453,
-18.2577352028925));
#69123=CARTESIAN_POINT('Ctrl Pts',(-20.6890778951259,-19.765352874987,-18.2624020880917));
#69124=CARTESIAN_POINT('Ctrl Pts',(-20.706553647153,-19.7220029411599,-18.2650452757123));
#69125=CARTESIAN_POINT('Ctrl Pts',(-20.7225805813239,-19.6781103714872,
-18.2676550109742));
#69126=CARTESIAN_POINT('Ctrl Pts',(-20.7225806448396,-19.6781101975385,
-18.0457833736847));
#69127=CARTESIAN_POINT('Ctrl Pts',(-20.6985992167088,-19.743787561633,-18.0412352539614));
#69128=CARTESIAN_POINT('Ctrl Pts',(-20.6713684492053,-19.8082648318828,
-18.0366093886528));
#69129=CARTESIAN_POINT('Ctrl Pts',(-20.6100512330559,-19.9354601153677,
-18.0272785871659));
#69130=CARTESIAN_POINT('Ctrl Pts',(-20.5759024792062,-19.9980201263964,
-18.022581895011));
#69131=CARTESIAN_POINT('Ctrl Pts',(-20.4894060415052,-20.1390620405839,
-18.0118326270559));
#69132=CARTESIAN_POINT('Ctrl Pts',(-20.4348362291936,-20.2160122140981,
-18.0058467969157));
#69133=CARTESIAN_POINT('Ctrl Pts',(-20.3617162823741,-20.3057696090812,
-17.9987328433445));
#69134=CARTESIAN_POINT('Ctrl Pts',(-20.3478652721742,-20.3222523079263,
-17.9974201993456));
#69135=CARTESIAN_POINT('Ctrl Pts',(-20.3291374813325,-20.34386038572,-17.9956903943503));
#69136=CARTESIAN_POINT('Ctrl Pts',(-20.3244833832923,-20.3491762691418,
-17.9952640983138));
#69137=CARTESIAN_POINT('Ctrl Pts',(-20.3152196348101,-20.3596509958889,
-17.9944225874072));
#69138=CARTESIAN_POINT('Ctrl Pts',(-20.3106111379901,-20.36481073788,-17.9940073320007));
#69139=CARTESIAN_POINT('Ctrl Pts',(-20.3016579801493,-20.3747364638025,
-17.9932070404168));
#69140=CARTESIAN_POINT('Ctrl Pts',(-20.297316677266,-20.3795053611674,-17.9928218694959));
#69141=CARTESIAN_POINT('Ctrl Pts',(-20.287266415397,-20.3904446832533,-17.9919367482262));
#69142=CARTESIAN_POINT('Ctrl Pts',(-20.2815423358339,-20.3966011165341,
-17.9914374480582));
#69143=CARTESIAN_POINT('Ctrl Pts',(-20.2661035773263,-20.4130089276943,
-17.9901034512516));
#69144=CARTESIAN_POINT('Ctrl Pts',(-20.2563226277584,-20.4231975699665,
-17.9892716094273));
#69145=CARTESIAN_POINT('Ctrl Pts',(-20.1714503993181,-20.5098547204957,
-17.9821641180485));
#69146=CARTESIAN_POINT('Ctrl Pts',(-20.0907499509967,-20.5806217774676,
-17.9761515338725));
#69147=CARTESIAN_POINT('Ctrl Pts',(-19.9106080183978,-20.7158657530999,
-17.9637760064709));
#69148=CARTESIAN_POINT('Ctrl Pts',(-19.8104277411408,-20.7787268359861,
-17.9574616387272));
#69149=CARTESIAN_POINT('Ctrl Pts',(-19.6539894100173,-20.8595308514712,
-17.9477550185748));
#69150=CARTESIAN_POINT('Ctrl Pts',(-19.6013774391923,-20.8840222273987,
-17.9445117946365));
#69151=CARTESIAN_POINT('Ctrl Pts',(-19.5207479925468,-20.9175984431095,
-17.9394791790417));
#69152=CARTESIAN_POINT('Ctrl Pts',(-19.4934356535838,-20.9283114470924,
-17.9377639594655));
#69153=CARTESIAN_POINT('Ctrl Pts',(-19.4593565842697,-20.9408679242767,
-17.9356005824247));
#69154=CARTESIAN_POINT('Ctrl Pts',(-19.4527902218378,-20.9432504635159,
-17.9351826874201));
#69155=CARTESIAN_POINT('Ctrl Pts',(-19.4423651837297,-20.9469748007534,
-17.9345173707888));
#69156=CARTESIAN_POINT('Ctrl Pts',(-19.4385141417142,-20.9483380256452,
-17.9342712024428));
#69157=CARTESIAN_POINT('Ctrl Pts',(-19.4312850051266,-20.9508735346393,
-17.9338083091325));
#69158=CARTESIAN_POINT('Ctrl Pts',(-19.4279078781634,-20.9520484098639,
-17.9335917403934));
#69159=CARTESIAN_POINT('Ctrl Pts',(-19.4201610685147,-20.9547214800779,
-17.9330942165664));
#69160=CARTESIAN_POINT('Ctrl Pts',(-19.4157894603182,-20.9562139280964,
-17.9328129266505));
#69161=CARTESIAN_POINT('Ctrl Pts',(-19.4022284822096,-20.9607940846542,
-17.9319387807732));
#69162=CARTESIAN_POINT('Ctrl Pts',(-19.3930229135797,-20.963832937933,-17.9313431595033));
#69163=CARTESIAN_POINT('Ctrl Pts',(-19.2884804287144,-20.9975489942562,
-17.9245564472342));
#69164=CARTESIAN_POINT('Ctrl Pts',(-19.1911133244138,-21.0214834811473,
-17.9180287429307));
#69165=CARTESIAN_POINT('Ctrl Pts',(-18.9235549270968,-21.067447692445,-17.9001409442158));
#69166=CARTESIAN_POINT('Ctrl Pts',(-18.7517479980882,-21.0758534142306,
-17.8887649758942));
#69167=CARTESIAN_POINT('Ctrl Pts',(-18.552076248789,-21.0613652529006,-17.8762269883954));
#69168=CARTESIAN_POINT('Ctrl Pts',(-18.5234034898055,-21.0586958151084,
-17.8744409990253));
#69169=CARTESIAN_POINT('Ctrl Pts',(-18.474140917004,-21.0530935915597,-17.8713968166211));
#69170=CARTESIAN_POINT('Ctrl Pts',(-18.4535240130681,-21.0504409194983,
-17.8701301536283));
#69171=CARTESIAN_POINT('Ctrl Pts',(-18.4240277792312,-21.0462032976491,
-17.8683279767776));
#69172=CARTESIAN_POINT('Ctrl Pts',(-18.4151148028715,-21.0448646550869,
-17.8677847202948));
#69173=CARTESIAN_POINT('Ctrl Pts',(-18.3997623697167,-21.0424585158982,
-17.8668511624229));
#69174=CARTESIAN_POINT('Ctrl Pts',(-18.3933188544185,-21.0414180909323,
-17.8664600091059));
#69175=CARTESIAN_POINT('Ctrl Pts',(-18.3809968245796,-21.0393699548819,
-17.8657132416991));
#69176=CARTESIAN_POINT('Ctrl Pts',(-18.3751175649468,-21.0383671703063,
-17.8653574753327));
#69177=CARTESIAN_POINT('Ctrl Pts',(-18.359853935092,-21.0356973305977,-17.8644352079534));
#69178=CARTESIAN_POINT('Ctrl Pts',(-18.3504763787318,-21.033991709847,-17.8638699372506));
#69179=CARTESIAN_POINT('Ctrl Pts',(-18.3186082338191,-21.0279728073589,
-17.8619532887333));
#69180=CARTESIAN_POINT('Ctrl Pts',(-18.2961757548717,-21.0233578654834,
-17.8606115141048));
#69181=CARTESIAN_POINT('Ctrl Pts',(-18.1013603417009,-20.9799729131537,
-17.8490127194019));
#69182=CARTESIAN_POINT('Ctrl Pts',(-17.9343872183227,-20.9201293438453,
-17.8395186852023));
#69183=CARTESIAN_POINT('Ctrl Pts',(-17.6999263807577,-20.8012713769272,
-17.8252130389209));
#69184=CARTESIAN_POINT('Ctrl Pts',(-17.6255313458058,-20.7576599270118,
-17.8204935063282));
#69185=CARTESIAN_POINT('Ctrl Pts',(-17.5227815950948,-20.6886788482865,
-17.8134260837131));
#69186=CARTESIAN_POINT('Ctrl Pts',(-17.4921228769797,-20.6668889949062,
-17.8112411213368));
#69187=CARTESIAN_POINT('Ctrl Pts',(-17.4560200241897,-20.6397539295148,
-17.8085539517204));
#69188=CARTESIAN_POINT('Ctrl Pts',(-17.450001601535,-20.6351798044172,-17.8081020740588));
#69189=CARTESIAN_POINT('Ctrl Pts',(-17.4406938917621,-20.6280267836449,
-17.8073968929144));
#69190=CARTESIAN_POINT('Ctrl Pts',(-17.4373874567062,-20.6254701613654,
-17.8071451346013));
#69191=CARTESIAN_POINT('Ctrl Pts',(-17.4312756465815,-20.6207153625459,
-17.8066773989691));
#69192=CARTESIAN_POINT('Ctrl Pts',(-17.4284682432846,-20.6185198870129,
-17.8064616125685));
#69193=CARTESIAN_POINT('Ctrl Pts',(-17.422141549697,-20.613546420914,-17.8059732076661));
#69194=CARTESIAN_POINT('Ctrl Pts',(-17.4186255528399,-20.6107643489616,
-17.8057003009175));
#69195=CARTESIAN_POINT('Ctrl Pts',(-17.4082960053871,-20.602537484983,-17.8048942318478));
#69196=CARTESIAN_POINT('Ctrl Pts',(-17.4015073313391,-20.5970618081456,
-17.8043589318196));
#69197=CARTESIAN_POINT('Ctrl Pts',(-17.3534129281117,-20.557776326218,-17.8005281183443));
#69198=CARTESIAN_POINT('Ctrl Pts',(-17.3133685901279,-20.5224596882375,
-17.7971354213675));
#69199=CARTESIAN_POINT('Ctrl Pts',(-17.262061964801,-20.4736412183802,-17.7925582246905));
#69200=CARTESIAN_POINT('Ctrl Pts',(-17.249568163393,-20.4614554235845,-17.791424360477));
#69201=CARTESIAN_POINT('Ctrl Pts',(-17.2028393473679,-20.4147373291041,
-17.7871140456336));
#69202=CARTESIAN_POINT('Ctrl Pts',(-17.1696475462279,-20.3791841500694,
-17.7839085274046));
#69203=CARTESIAN_POINT('Ctrl Pts',(-17.0658627852009,-20.2600413371745,
-17.7734710134909));
#69204=CARTESIAN_POINT('Ctrl Pts',(-17.0005103316433,-20.1721110369868,
-17.7662381123081));
#69205=CARTESIAN_POINT('Ctrl Pts',(-16.9128955757416,-20.0328811380464,
-17.7556642494986));
#69206=CARTESIAN_POINT('Ctrl Pts',(-16.8853777886072,-19.9851128202315,
-17.7521749114311));
#69207=CARTESIAN_POINT('Ctrl Pts',(-16.8438032680044,-19.9059507927004,
-17.7466170589514));
#69208=CARTESIAN_POINT('Ctrl Pts',(-16.8285928973241,-19.8751954234934,
-17.7445101009141));
#69209=CARTESIAN_POINT('Ctrl Pts',(-16.809581353943,-19.8342803978335,-17.7417734717013));
#69210=CARTESIAN_POINT('Ctrl Pts',(-16.8051017923191,-19.8244434290454,
-17.7411204570575));
#69211=CARTESIAN_POINT('Ctrl Pts',(-16.7978870878274,-19.808272955516,-17.7400549450428));
#69212=CARTESIAN_POINT('Ctrl Pts',(-16.7951072574144,-19.8019597152397,
-17.7396409181602));
#69213=CARTESIAN_POINT('Ctrl Pts',(-16.7897852784013,-19.7897110513713,
-17.7388414016324));
#69214=CARTESIAN_POINT('Ctrl Pts',(-16.7872393324841,-19.7837773705202,
-17.7384557856285));
#69215=CARTESIAN_POINT('Ctrl Pts',(-16.7814224725198,-19.7700473571059,
-17.737567371586));
#69216=CARTESIAN_POINT('Ctrl Pts',(-16.7781710218343,-19.7622428590363,
-17.7370652395822));
#69217=CARTESIAN_POINT('Ctrl Pts',(-16.7695501595302,-19.7411958012982,
-17.7357186539877));
#69218=CARTESIAN_POINT('Ctrl Pts',(-16.7642678686016,-19.7279178654694,
-17.734877141636));
#69219=CARTESIAN_POINT('Ctrl Pts',(-16.7170425207028,-19.6056179137501,
-17.7271967971292));
#69220=CARTESIAN_POINT('Ctrl Pts',(-16.6840528963727,-19.4933464543303,
-17.7206745015522));
#69221=CARTESIAN_POINT('Ctrl Pts',(-16.6276808696708,-19.2195486913437,
-17.705371054411));
#69222=CARTESIAN_POINT('Ctrl Pts',(-16.6133548999859,-19.0569528627794,
-17.6967728845433));
#69223=CARTESIAN_POINT('Ctrl Pts',(-16.6186718954416,-18.8618019649981,
-17.6855640193953));
#69224=CARTESIAN_POINT('Ctrl Pts',(-16.6203088644817,-18.8292881553707,
-17.6836654624941));
#69225=CARTESIAN_POINT('Ctrl Pts',(-16.623225504645,-18.789603923699,-17.6812962694845));
#69226=CARTESIAN_POINT('Ctrl Pts',(-16.6237934346789,-18.7823836562483,
-17.6808631038559));
#69227=CARTESIAN_POINT('Ctrl Pts',(-16.6247417335092,-18.7710705653313,
-17.6801808945602));
#69228=CARTESIAN_POINT('Ctrl Pts',(-16.6250969981053,-18.7669756150441,
-17.6799332381386));
#69229=CARTESIAN_POINT('Ctrl Pts',(-16.6257832670682,-18.7593241969135,
-17.6794691026115));
#69230=CARTESIAN_POINT('Ctrl Pts',(-16.6261113472134,-18.7557675233129,
-17.679252789121));
#69231=CARTESIAN_POINT('Ctrl Pts',(-16.6268807041034,-18.747651635749,-17.6787579065834));
#69232=CARTESIAN_POINT('Ctrl Pts',(-16.6273277763972,-18.743093029074,-17.6784790160038));
#69233=CARTESIAN_POINT('Ctrl Pts',(-16.6287470647711,-18.7290891721719,
-17.6776195212924));
#69234=CARTESIAN_POINT('Ctrl Pts',(-16.6297680199109,-18.7196491344887,
-17.6770362812199));
#69235=CARTESIAN_POINT('Ctrl Pts',(-16.6395752256174,-18.6343414109738,
-17.6717327447863));
#69236=CARTESIAN_POINT('Ctrl Pts',(-16.6523967615574,-18.559001924081,-17.66681493842));
#69237=CARTESIAN_POINT('Ctrl Pts',(-16.6708311433045,-18.4775803266455,
-17.6613539437278));
#69238=CARTESIAN_POINT('Ctrl Pts',(-16.6724394045865,-18.4706397731387,
-17.6608872430014));
#69239=CARTESIAN_POINT('Ctrl Pts',(-16.7048775657934,-18.3337957051517,
-17.6516633272659));
#69240=CARTESIAN_POINT('Ctrl Pts',(-16.7478961666825,-18.2070770008716,
-17.6427531064208));
#69241=CARTESIAN_POINT('Ctrl Pts',(-16.8280081432266,-18.0285576436559,
-17.6301080429714));
#69242=CARTESIAN_POINT('Ctrl Pts',(-16.8559365444506,-17.9730058488077,
-17.6261544149705));
#69243=CARTESIAN_POINT('Ctrl Pts',(-16.9045255954434,-17.8861147889895,
-17.6199504218185));
#69244=CARTESIAN_POINT('Ctrl Pts',(-16.9236428699102,-17.853958460988,-17.6176495302413));
#69245=CARTESIAN_POINT('Ctrl Pts',(-16.9495530746944,-17.8128939930676,
-17.6147027916065));
#69246=CARTESIAN_POINT('Ctrl Pts',(-16.9555774871667,-17.8035111243199,
-17.6140288856109));
#69247=CARTESIAN_POINT('Ctrl Pts',(-16.9654896543488,-17.7883382002817,
-17.6129380108901));
#69248=CARTESIAN_POINT('Ctrl Pts',(-16.9693323245552,-17.7825190793135,
-17.61251936986));
#69249=CARTESIAN_POINT('Ctrl Pts',(-16.9767732295691,-17.7713711769132,
-17.6117168028945));
#69250=CARTESIAN_POINT('Ctrl Pts',(-16.9803671205189,-17.7660396018274,
-17.611332719701));
#69251=CARTESIAN_POINT('Ctrl Pts',(-16.9886456148864,-17.753878278721,-17.6104560097564));
#69252=CARTESIAN_POINT('Ctrl Pts',(-16.9933461366148,-17.747059453959,-17.6099639926086));
#69253=CARTESIAN_POINT('Ctrl Pts',(-17.0059270941754,-17.7290361134634,
-17.6086621888729));
#69254=CARTESIAN_POINT('Ctrl Pts',(-17.013876549892,-17.7178800847709,-17.6078550418735));
#69255=CARTESIAN_POINT('Ctrl Pts',(-17.0744631666554,-17.63457744702,-17.6018159181769));
#69256=CARTESIAN_POINT('Ctrl Pts',(-17.1315133690548,-17.565744587087,-17.5967623212738));
#69257=CARTESIAN_POINT('Ctrl Pts',(-17.2884850846914,-17.3990419468733,
-17.5840804871437));
#69258=CARTESIAN_POINT('Ctrl Pts',(-17.3940439899097,-17.3070962886841,
-17.5766518411665));
#69259=CARTESIAN_POINT('Ctrl Pts',(-17.5534533491994,-17.1938409483206,
-17.5658553959733));
#69260=CARTESIAN_POINT('Ctrl Pts',(-17.6002833114379,-17.1632855893545,
-17.5627248869781));
#69261=CARTESIAN_POINT('Ctrl Pts',(-17.6728937552751,-17.1199067468825,
-17.5578472689787));
#69262=CARTESIAN_POINT('Ctrl Pts',(-17.6978189655542,-17.1056953580475,
-17.5561688116792));
#69263=CARTESIAN_POINT('Ctrl Pts',(-17.7291388095643,-17.0886719483782,
-17.5540449891703));
#69264=CARTESIAN_POINT('Ctrl Pts',(-17.7352700482102,-17.085378474266,-17.5536285338077));
#69265=CARTESIAN_POINT('Ctrl Pts',(-17.744992736391,-17.0802174222796,-17.5529668666106));
#69266=CARTESIAN_POINT('Ctrl Pts',(-17.7485735562737,-17.0783297757871,
-17.5527229072413));
#69267=CARTESIAN_POINT('Ctrl Pts',(-17.7553337898359,-17.0747908255488,
-17.5522617854239));
#69268=CARTESIAN_POINT('Ctrl Pts',(-17.7585119892116,-17.073137318574,-17.5520447650108));
#69269=CARTESIAN_POINT('Ctrl Pts',(-17.7657835211257,-17.0693776157916,
-17.5515477175492));
#69270=CARTESIAN_POINT('Ctrl Pts',(-17.7698795310851,-17.0672767014806,
-17.5512673631174));
#69271=CARTESIAN_POINT('Ctrl Pts',(-17.7807630372948,-17.0617391254021,
-17.5505215178186));
#69272=CARTESIAN_POINT('Ctrl Pts',(-17.7875621910878,-17.0583257009259,
-17.5500546314522));
#69273=CARTESIAN_POINT('Ctrl Pts',(-17.8350485104516,-17.0348054468173,
-17.5467880612411));
#69274=CARTESIAN_POINT('Ctrl Pts',(-17.8763515972135,-17.0159764254801,
-17.5439176359258));
#69275=CARTESIAN_POINT('Ctrl Pts',(-17.9235895562848,-16.9962500874831,
-17.5406275739431));
#69276=CARTESIAN_POINT('Ctrl Pts',(-17.9289641176092,-16.9940316563879,
-17.5402531364634));
#69277=CARTESIAN_POINT('Ctrl Pts',(-18.0801760273008,-16.9323445148577,
-17.5297166909062));
#69278=CARTESIAN_POINT('Ctrl Pts',(-18.2321878966764,-16.8893118555842,
-17.5191262198398));
#69279=CARTESIAN_POINT('Ctrl Pts',(-18.489180696128,-16.8466827395006,-17.502214494249));
#69280=CARTESIAN_POINT('Ctrl Pts',(-18.5918943469089,-16.8372639153502,
-17.495695274456));
#69281=CARTESIAN_POINT('Ctrl Pts',(-18.7097046581973,-16.835087626326,-17.4885096620398));
#69282=CARTESIAN_POINT('Ctrl Pts',(-18.7245123588162,-16.8349694703209,
-17.4876115365446));
#69283=CARTESIAN_POINT('Ctrl Pts',(-18.7470890134317,-16.8350262094805,
-17.4862496405256));
#69284=CARTESIAN_POINT('Ctrl Pts',(-18.7548575580758,-16.8350884957562,
-17.4857823586322));
#69285=CARTESIAN_POINT('Ctrl Pts',(-18.7689864733627,-16.8352795616905,
-17.4849348837307));
#69286=CARTESIAN_POINT('Ctrl Pts',(-18.7753469141363,-16.8353942499052,
-17.4845542540677));
#69287=CARTESIAN_POINT('Ctrl Pts',(-18.7890725678174,-16.8357036373795,
-17.483734725267));
#69288=CARTESIAN_POINT('Ctrl Pts',(-18.7964374932963,-16.8359081202126,
-17.4832961374704));
#69289=CARTESIAN_POINT('Ctrl Pts',(-18.8163931797336,-16.8365664528046,
-17.482110806357));
#69290=CARTESIAN_POINT('Ctrl Pts',(-18.8289813257046,-16.8370942605501,
-17.4813663839479));
#69291=CARTESIAN_POINT('Ctrl Pts',(-18.890049833593,-16.8402011485294,-17.4777700938631));
#69292=CARTESIAN_POINT('Ctrl Pts',(-18.9384386531467,-16.8443351053112,
-17.4749672011889));
#69293=CARTESIAN_POINT('Ctrl Pts',(-19.0271592539814,-16.8549993479368,
-17.4698883422315));
#69294=CARTESIAN_POINT('Ctrl Pts',(-19.0675251277346,-16.8610396182918,
-17.4676006621723));
#69295=CARTESIAN_POINT('Ctrl Pts',(-19.240032468628,-16.8919764056235,-17.4578739050451));
#69296=CARTESIAN_POINT('Ctrl Pts',(-19.3698060735372,-16.9282618728386,
-17.4507040792665));
#69297=CARTESIAN_POINT('Ctrl Pts',(-19.5537918318525,-16.9991648854428,
-17.4398677829608));
#69298=CARTESIAN_POINT('Ctrl Pts',(-19.6112870808457,-17.0243097083801,
-17.4363742441128));
#69299=CARTESIAN_POINT('Ctrl Pts',(-19.6953392890889,-17.065608575186,-17.4309875260399));
#69300=CARTESIAN_POINT('Ctrl Pts',(-19.7227978722138,-17.0798556740738,
-17.4291811433687));
#69301=CARTESIAN_POINT('Ctrl Pts',(-19.7561871479493,-17.0981194064623,
-17.4269145719479));
#69302=CARTESIAN_POINT('Ctrl Pts',(-19.7624240619938,-17.101572004657,-17.4264881299539));
#69303=CARTESIAN_POINT('Ctrl Pts',(-19.7722074760035,-17.1070525952048,
-17.4258141834715));
#69304=CARTESIAN_POINT('Ctrl Pts',(-19.775765812932,-17.1090595017616,-17.425568011292));
#69305=CARTESIAN_POINT('Ctrl Pts',(-19.782427697071,-17.1128422716382,-17.4251051148299));
#69306=CARTESIAN_POINT('Ctrl Pts',(-19.7855325616823,-17.1146157024669,
-17.4248885467968));
#69307=CARTESIAN_POINT('Ctrl Pts',(-19.7926381809225,-17.1186981864264,
-17.4243910299956));
#69308=CARTESIAN_POINT('Ctrl Pts',(-19.7966358694327,-17.1210124670493,
-17.4241097464343));
#69309=CARTESIAN_POINT('Ctrl Pts',(-19.8089993446969,-17.1282238685638,
-17.4232356395496));
#69310=CARTESIAN_POINT('Ctrl Pts',(-19.8173389552097,-17.1331652992591,
-17.422640051266));
#69311=CARTESIAN_POINT('Ctrl Pts',(-19.9078157475782,-17.1876180976281,
-17.4161156738663));
#69312=CARTESIAN_POINT('Ctrl Pts',(-19.9865225158485,-17.2425936984073,
-17.4098777262563));
#69313=CARTESIAN_POINT('Ctrl Pts',(-20.1599394870345,-17.3821460663,-17.3952247396011));
#69314=CARTESIAN_POINT('Ctrl Pts',(-20.2513337290229,-17.470295712805,-17.3867948646594));
#69315=CARTESIAN_POINT('Ctrl Pts',(-20.3724501451461,-17.6101480943695,
-17.3748732318351));
#69316=CARTESIAN_POINT('Ctrl Pts',(-20.4087696807897,-17.6557620235852,
-17.3711748599224));
#69317=CARTESIAN_POINT('Ctrl Pts',(-20.4642422251247,-17.7316611235917,
-17.3653244509211));
#69318=CARTESIAN_POINT('Ctrl Pts',(-20.4845888555995,-17.7610323120921,
-17.3631287336968));
#69319=CARTESIAN_POINT('Ctrl Pts',(-20.510199220617,-17.8000774174205,-17.3602956709622));
#69320=CARTESIAN_POINT('Ctrl Pts',(-20.5161437329624,-17.809295738289,-17.3596328756309));
#69321=CARTESIAN_POINT('Ctrl Pts',(-20.5257284581396,-17.8244157673421,
-17.3585554921701));
#69322=CARTESIAN_POINT('Ctrl Pts',(-20.5294117393818,-17.8302898068951,
-17.3581393082602));
#69323=CARTESIAN_POINT('Ctrl Pts',(-20.5364622258217,-17.8416575121252,
-17.3573384123058));
#69324=CARTESIAN_POINT('Ctrl Pts',(-20.5398333326735,-17.8471486561911,
-17.3569535592604));
#69325=CARTESIAN_POINT('Ctrl Pts',(-20.5475262651513,-17.8598088279156,
-17.3560708381274));
#69326=CARTESIAN_POINT('Ctrl Pts',(-20.5518307630405,-17.8669882992394,
-17.355573608656));
#69327=CARTESIAN_POINT('Ctrl Pts',(-20.5632211500836,-17.8862443847782,
-17.3542487915019));
#69328=CARTESIAN_POINT('Ctrl Pts',(-20.5702300778545,-17.8983662104354,
-17.3534239964177));
#69329=CARTESIAN_POINT('Ctrl Pts',(-20.6269882510109,-17.9988153189563,
-17.346662346183));
#69330=CARTESIAN_POINT('Ctrl Pts',(-20.6704578060138,-18.090547429438,-17.3409590585524));
#69331=CARTESIAN_POINT('Ctrl Pts',(-20.7617037772607,-18.3253034172797,
-17.3270884327748));
#69332=CARTESIAN_POINT('Ctrl Pts',(-20.801104883465,-18.4709561073493,-17.3191198091754));
#69333=CARTESIAN_POINT('Ctrl Pts',(-20.8309456096504,-18.6586173383895,
-17.3084711081853));
#69334=CARTESIAN_POINT('Ctrl Pts',(-20.8360618097048,-18.6978542603052,
-17.3062221383147));
#69335=CARTESIAN_POINT('Ctrl Pts',(-20.8416060205161,-18.7522165428395,
-17.3030474899831));
#69336=CARTESIAN_POINT('Ctrl Pts',(-20.8429760806296,-18.7672395279161,
-17.3021640059745));
#69337=CARTESIAN_POINT('Ctrl Pts',(-20.8450676747903,-18.7932443154418,
-17.3006220664936));
#69338=CARTESIAN_POINT('Ctrl Pts',(-20.8458643547452,-18.8042196548609,
-17.299967406966));
#69339=CARTESIAN_POINT('Ctrl Pts',(-20.8468897381119,-18.8200544988783,
-17.2990166524564));
#69340=CARTESIAN_POINT('Ctrl Pts',(-20.8471873278301,-18.8249095711491,
-17.298724300212));
#69341=CARTESIAN_POINT('Ctrl Pts',(-20.8476764826059,-18.833367196857,-17.2982134803064));
#69342=CARTESIAN_POINT('Ctrl Pts',(-20.8478755777288,-18.8369693221484,
-17.2979954343208));
#69343=CARTESIAN_POINT('Ctrl Pts',(-20.8482735902507,-18.8445206030594,
-17.2975372912288));
#69344=CARTESIAN_POINT('Ctrl Pts',(-20.8484706504524,-18.8484697967728,
-17.2972970960155));
#69345=CARTESIAN_POINT('Ctrl Pts',(-20.8489642020208,-18.8589506832107,
-17.296658100317));
#69346=CARTESIAN_POINT('Ctrl Pts',(-20.8492414963272,-18.8654831761259,
-17.2962582484209));
#69347=CARTESIAN_POINT('Ctrl Pts',(-20.8502933311974,-18.8933033080977,
-17.2945489587838));
#69348=CARTESIAN_POINT('Ctrl Pts',(-20.8507767751215,-18.9145998759567,
-17.2932244674539));
#69349=CARTESIAN_POINT('Ctrl Pts',(-20.8509781231638,-18.9410730908942,
-17.2915611068256));
#69350=CARTESIAN_POINT('Ctrl Pts',(-20.8509985064325,-18.9462471151322,
-17.2912352096919));
#69351=CARTESIAN_POINT('Ctrl Pts',(-20.851013182946,-18.9999278666397,-17.287846021773));
#69352=CARTESIAN_POINT('Ctrl Pts',(-20.8493592891962,-19.0484176143119,
-17.2847171782446));
#69353=CARTESIAN_POINT('Ctrl Pts',(-20.832613863639,-19.2926578376087,-17.2687464657044));
#69354=CARTESIAN_POINT('Ctrl Pts',(-20.7920024742,-19.485740026347,-17.2555538234773));
#69355=CARTESIAN_POINT('Ctrl Pts',(-20.724436348768,-19.6730128285728,-17.243039546343));
#69356=CARTESIAN_POINT('Ctrl Pts',(-20.7235109086517,-19.6755625069505,
-17.2428691976168));
#69357=CARTESIAN_POINT('Ctrl Pts',(-20.7225805822089,-19.6781103690637,
-17.242699000807));
#69358=CARTESIAN_POINT('Origin',(-18.734,-18.952,0.));
#69359=CARTESIAN_POINT('',(-20.7225805882177,-19.6781103526075,-16.4437314133151));
#69360=CARTESIAN_POINT('',(-20.7225805820307,-19.6781103695518,-16.6645990581914));
#69361=CARTESIAN_POINT('',(-20.7225805821191,-19.6781103693095,0.));
#69362=CARTESIAN_POINT('',(-20.8509997150765,-18.9530983468555,-16.7126937598086));
#69363=CARTESIAN_POINT('Ctrl Pts',(-20.7225805820307,-19.6781103695518,
-16.6645990581914));
#69364=CARTESIAN_POINT('Ctrl Pts',(-20.724617954831,-19.6725306668522,-16.6649758082994));
#69365=CARTESIAN_POINT('Ctrl Pts',(-20.7266318565325,-19.6669423541826,
-16.6653535212313));
#69366=CARTESIAN_POINT('Ctrl Pts',(-20.755309382627,-19.586303477032,-16.6708086650019));
#69367=CARTESIAN_POINT('Ctrl Pts',(-20.7777386604433,-19.5098199607894,
-16.6760396990613));
#69368=CARTESIAN_POINT('Ctrl Pts',(-20.8323931999723,-19.275182842516,-16.6919443777136));
#69369=CARTESIAN_POINT('Ctrl Pts',(-20.8509160191727,-19.1144173361511,
-16.7026019321524));
#69370=CARTESIAN_POINT('Ctrl Pts',(-20.8509997150765,-18.9530983468555,
-16.7126937598086));
#69371=CARTESIAN_POINT('Ctrl Pts',(-20.8509997162488,-18.9530960850687,
-16.7126939013019));
#69372=CARTESIAN_POINT('Ctrl Pts',(-20.8510131380886,-18.9271728863108,
-16.7143156094758));
#69373=CARTESIAN_POINT('Ctrl Pts',(-20.8505504063366,-18.9012505606405,
-16.7159233010165));
#69374=CARTESIAN_POINT('Ctrl Pts',(-20.8489736678282,-18.8577355730853,
-16.7185990754188));
#69375=CARTESIAN_POINT('Ctrl Pts',(-20.8481159277891,-18.8401372666953,
-16.7196748919229));
#69376=CARTESIAN_POINT('Ctrl Pts',(-20.8465415700014,-18.8144384493095,
-16.7212369878273));
#69377=CARTESIAN_POINT('Ctrl Pts',(-20.8459978380121,-18.8063284505031,
-16.7217286535888));
#69378=CARTESIAN_POINT('Ctrl Pts',(-20.8449526632468,-18.7919779884224,
-16.7225963976334));
#69379=CARTESIAN_POINT('Ctrl Pts',(-20.8444702241123,-18.7857362784398,
-16.7229730681296));
#69380=CARTESIAN_POINT('Ctrl Pts',(-20.8434611317316,-18.7733936435573,
-16.723716452697));
#69381=CARTESIAN_POINT('Ctrl Pts',(-20.8429356807584,-18.7672926842432,
-16.7240832007903));
#69382=CARTESIAN_POINT('Ctrl Pts',(-20.8418361311527,-18.7551427884005,
-16.7248121932608));
#69383=CARTESIAN_POINT('Ctrl Pts',(-20.8412624475386,-18.749093874097,-16.7251744470071));
#69384=CARTESIAN_POINT('Ctrl Pts',(-20.8398285557079,-18.7346373542702,
-16.7260386236379));
#69385=CARTESIAN_POINT('Ctrl Pts',(-20.8389440230463,-18.726232223773,-16.7265397777864));
#69386=CARTESIAN_POINT('Ctrl Pts',(-20.8360988459888,-18.7006681331952,
-16.7280602738497));
#69387=CARTESIAN_POINT('Ctrl Pts',(-20.8339785134003,-18.6835274037956,
-16.729074601943));
#69388=CARTESIAN_POINT('Ctrl Pts',(-20.8260337980322,-18.6251728964754,
-16.7325119101018));
#69389=CARTESIAN_POINT('Ctrl Pts',(-20.8192037210801,-18.584104449838,-16.7349036449326));
#69390=CARTESIAN_POINT('Ctrl Pts',(-20.7779734452175,-18.374576171713,-16.7470134350623));
#69391=CARTESIAN_POINT('Ctrl Pts',(-20.72435859662,-18.2105701549565,-16.7561209992149));
#69392=CARTESIAN_POINT('Ctrl Pts',(-20.6249327975613,-17.9980645897377,
-16.769015153791));
#69393=CARTESIAN_POINT('Ctrl Pts',(-20.5958562709737,-17.942490371582,-16.7725069951293));
#69394=CARTESIAN_POINT('Ctrl Pts',(-20.5488219970765,-17.8615568214716,
-16.7778913461385));
#69395=CARTESIAN_POINT('Ctrl Pts',(-20.5327016305221,-17.8351663400157,
-16.7796971488983));
#69396=CARTESIAN_POINT('Ctrl Pts',(-20.512161980929,-17.8031397910929,-16.7819630741043));
#69397=CARTESIAN_POINT('Ctrl Pts',(-20.5082836580815,-17.7971591852528,
-16.7823894725882));
#69398=CARTESIAN_POINT('Ctrl Pts',(-20.5021352894321,-17.7877821137658,
-16.7830633655851));
#69399=CARTESIAN_POINT('Ctrl Pts',(-20.4998854481123,-17.7843723744879,
-16.7833095281413));
#69400=CARTESIAN_POINT('Ctrl Pts',(-20.4956478280947,-17.7779903255335,
-16.7837724166871));
#69401=CARTESIAN_POINT('Ctrl Pts',(-20.4936623832969,-17.7750165327831,
-16.7839889864883));
#69402=CARTESIAN_POINT('Ctrl Pts',(-20.4890946293522,-17.7682123576569,
-16.7844865209106));
#69403=CARTESIAN_POINT('Ctrl Pts',(-20.4865073177234,-17.7643853989878,
-16.7847678204131));
#69404=CARTESIAN_POINT('Ctrl Pts',(-20.4784512076748,-17.7525530530541,
-16.7856420251302));
#69405=CARTESIAN_POINT('Ctrl Pts',(-20.4729400170964,-17.7445768748147,
-16.7862376961793));
#69406=CARTESIAN_POINT('Ctrl Pts',(-20.4106714911215,-17.6557681447812,
-16.7929390766375));
#69407=CARTESIAN_POINT('Ctrl Pts',(-20.3483849201451,-17.5789737756689,
-16.7993723401165));
#69408=CARTESIAN_POINT('Ctrl Pts',(-20.1664592961763,-17.3842341394247,
-16.8169267902971));
#69409=CARTESIAN_POINT('Ctrl Pts',(-20.0377573445236,-17.2756758282441,
-16.8280724934787));
#69410=CARTESIAN_POINT('Ctrl Pts',(-19.8712093187778,-17.166099638103,-16.8405986465004));
#69411=CARTESIAN_POINT('Ctrl Pts',(-19.844456895574,-17.1493434088667,-16.8425612660863));
#69412=CARTESIAN_POINT('Ctrl Pts',(-19.8041716999014,-17.1253483069514,
-16.8454447891522));
#69413=CARTESIAN_POINT('Ctrl Pts',(-19.790919729861,-17.1176487307524,-16.8463820970399));
#69414=CARTESIAN_POINT('Ctrl Pts',(-19.7666473131505,-17.1038964952453,
-16.8480787964603));
#69415=CARTESIAN_POINT('Ctrl Pts',(-19.7556544262716,-17.0977968607478,
-16.8488398499652));
#69416=CARTESIAN_POINT('Ctrl Pts',(-19.7382624433009,-17.0883481842936,
-16.8500325341717));
#69417=CARTESIAN_POINT('Ctrl Pts',(-19.7318995612018,-17.0849334203156,
-16.850466505087));
#69418=CARTESIAN_POINT('Ctrl Pts',(-19.7254731392043,-17.0815267933058,
-16.850902449066));
#69419=CARTESIAN_POINT('Ctrl Pts',(-19.7254270071262,-17.0815023410157,
-16.8509055783682));
#69420=CARTESIAN_POINT('Ctrl Pts',(-19.7253331168546,-17.0814525789632,
-16.8509119470292));
#69421=CARTESIAN_POINT('Ctrl Pts',(-19.7252853576638,-17.0814272688287,
-16.8509151864468));
#69422=CARTESIAN_POINT('Ctrl Pts',(-19.7251881538843,-17.081375760146,-16.8509217793332));
#69423=CARTESIAN_POINT('Ctrl Pts',(-19.7251387082889,-17.0813495612324,
-16.8509251328607));
#69424=CARTESIAN_POINT('Ctrl Pts',(-19.7250380701728,-17.0812962429013,
-16.8509319581113));
#69425=CARTESIAN_POINT('Ctrl Pts',(-19.7249868767742,-17.081269123199,-16.8509354298838));
#69426=CARTESIAN_POINT('Ctrl Pts',(-19.7248826792599,-17.0812139300446,
-16.8509424959198));
#69427=CARTESIAN_POINT('Ctrl Pts',(-19.7248296743174,-17.0811858563479,
-16.8509460902286));
#69428=CARTESIAN_POINT('Ctrl Pts',(-19.7247217876403,-17.081128720796,-16.850953405785));
#69429=CARTESIAN_POINT('Ctrl Pts',(-19.7246669050773,-17.0810996587096,
-16.8509571270772));
#69430=CARTESIAN_POINT('Ctrl Pts',(-19.7245551946518,-17.0810405107319,
-16.8509647012105));
#69431=CARTESIAN_POINT('Ctrl Pts',(-19.724498366005,-17.0810104246481,-16.8509685540922));
#69432=CARTESIAN_POINT('Ctrl Pts',(-19.7243826923224,-17.0809491917159,
-16.8509763961865));
#69433=CARTESIAN_POINT('Ctrl Pts',(-19.7243238466558,-17.0809180447727,
-16.8509803854284));
#69434=CARTESIAN_POINT('Ctrl Pts',(-19.7242040653581,-17.0808546519042,
-16.8509885051904));
#69435=CARTESIAN_POINT('Ctrl Pts',(-19.7241431290711,-17.0808224058882,
-16.8509926357406));
#69436=CARTESIAN_POINT('Ctrl Pts',(-19.7240190902981,-17.0807567753119,
-16.8510010432431));
#69437=CARTESIAN_POINT('Ctrl Pts',(-19.7239559872454,-17.0807233907268,
-16.8510053202185));
#69438=CARTESIAN_POINT('Ctrl Pts',(-19.7238275359928,-17.0806554420805,
-16.8510140258757));
#69439=CARTESIAN_POINT('Ctrl Pts',(-19.723762187258,-17.0806208780316,-16.8510184545774));
#69440=CARTESIAN_POINT('Ctrl Pts',(-19.7236291608479,-17.0805505270352,
-16.8510274693158));
#69441=CARTESIAN_POINT('Ctrl Pts',(-19.7235614857846,-17.0805147417862,
-16.8510320551578));
#69442=CARTESIAN_POINT('Ctrl Pts',(-19.7234348766143,-17.0804478021219,
-16.851040634041));
#69443=CARTESIAN_POINT('Ctrl Pts',(-19.7233759417252,-17.0804166461579,
-16.8510446271985));
#69444=CARTESIAN_POINT('Ctrl Pts',(-19.7232483209136,-17.0803491870531,
-16.8510532737683));
#69445=CARTESIAN_POINT('Ctrl Pts',(-19.7231796333278,-17.0803128843086,
-16.8510579272222));
#69446=CARTESIAN_POINT('Ctrl Pts',(-19.7230309106786,-17.0802342919276,
-16.8510680023154));
#69447=CARTESIAN_POINT('Ctrl Pts',(-19.7229508740339,-17.0801920031847,
-16.8510734239655));
#69448=CARTESIAN_POINT('Ctrl Pts',(-19.7227776033407,-17.0801004668387,
-16.8510851604592));
#69449=CARTESIAN_POINT('Ctrl Pts',(-19.7226843676137,-17.0800512206916,
-16.8510914752859));
#69450=CARTESIAN_POINT('Ctrl Pts',(-19.7224825586956,-17.0799446465905,
-16.8511051426651));
#69451=CARTESIAN_POINT('Ctrl Pts',(-19.7223739837106,-17.0798873208594,
-16.8511124951622));
#69452=CARTESIAN_POINT('Ctrl Pts',(-19.7221390256547,-17.0797632931704,
-16.8511284046293));
#69453=CARTESIAN_POINT('Ctrl Pts',(-19.7220126410725,-17.0796965946987,
-16.8511369614626));
#69454=CARTESIAN_POINT('Ctrl Pts',(-19.721726714621,-17.0795457362701,-16.8511563179702));
#69455=CARTESIAN_POINT('Ctrl Pts',(-19.7215671687158,-17.0794615838891,
-16.8511671173765));
#69456=CARTESIAN_POINT('Ctrl Pts',(-19.7156957081335,-17.0763656450527,
-16.851564493651));
#69457=CARTESIAN_POINT('Ctrl Pts',(-19.7099700060516,-17.0733799624352,
-16.8519501429257));
#69458=CARTESIAN_POINT('Ctrl Pts',(-19.6967131573479,-17.0665441091715,
-16.8528388002148));
#69459=CARTESIAN_POINT('Ctrl Pts',(-19.6891723860932,-17.0627127651934,
-16.8533411410233));
#69460=CARTESIAN_POINT('Ctrl Pts',(-19.6688197882023,-17.0525249399193,
-16.8546886564778));
#69461=CARTESIAN_POINT('Ctrl Pts',(-19.6559660359483,-17.0462528541833,
-16.8555308834503));
#69462=CARTESIAN_POINT('Ctrl Pts',(-19.5375050260952,-16.9899279627722,
-16.8632151229833));
#69463=CARTESIAN_POINT('Ctrl Pts',(-19.4279800945321,-16.9485669714425,
-16.8697402894631));
#69464=CARTESIAN_POINT('Ctrl Pts',(-19.1589136982039,-16.8716904318624,
-16.88505936679));
#69465=CARTESIAN_POINT('Ctrl Pts',(-18.997615162597,-16.8451695239618,-16.893669571053));
#69466=CARTESIAN_POINT('Ctrl Pts',(-18.8026567586164,-16.8358674841518,
-16.9048794202438));
#69467=CARTESIAN_POINT('Ctrl Pts',(-18.7703909923844,-16.8350668374245,
-16.906762104127));
#69468=CARTESIAN_POINT('Ctrl Pts',(-18.7308980986525,-16.8349899487626,
-16.9091136371913));
#69469=CARTESIAN_POINT('Ctrl Pts',(-18.7236747143635,-16.8350128569384,
-16.9095456714452));
#69470=CARTESIAN_POINT('Ctrl Pts',(-18.7123456960382,-16.8351067689632,
-16.9102264906488));
#69471=CARTESIAN_POINT('Ctrl Pts',(-18.7082398322799,-16.8351527514745,
-16.9104738976636));
#69472=CARTESIAN_POINT('Ctrl Pts',(-18.7005620656589,-16.8352610772688,
-16.9109378224223));
#69473=CARTESIAN_POINT('Ctrl Pts',(-18.6969901780054,-16.835320516735,-16.911154176116));
#69474=CARTESIAN_POINT('Ctrl Pts',(-18.6888324315153,-16.8354769242404,
-16.9116494895984));
#69475=CARTESIAN_POINT('Ctrl Pts',(-18.6842467421793,-16.8355797553682,
-16.9119287730984));
#69476=CARTESIAN_POINT('Ctrl Pts',(-18.6701369837262,-16.8359420398154,
-16.9127906574356));
#69477=CARTESIAN_POINT('Ctrl Pts',(-18.6606144566246,-16.8362508820904,
-16.9133759151013));
#69478=CARTESIAN_POINT('Ctrl Pts',(-18.5315880865436,-16.8413076614831,
-16.9213515081989));
#69479=CARTESIAN_POINT('Ctrl Pts',(-18.4127068930046,-16.8561095355057,
-16.9292186583405));
#69480=CARTESIAN_POINT('Ctrl Pts',(-18.1891141765261,-16.9034239902712,
-16.9443169102164));
#69481=CARTESIAN_POINT('Ctrl Pts',(-18.0843942606154,-16.9341843275615,
-16.9515201160467));
#69482=CARTESIAN_POINT('Ctrl Pts',(-17.9123465694994,-16.9995128164646,
-16.9633445893002));
#69483=CARTESIAN_POINT('Ctrl Pts',(-17.843650472363,-17.0298656583292,-16.9680660297628));
#69484=CARTESIAN_POINT('Ctrl Pts',(-17.7599286851908,-17.0723117678669,
-16.9738163683881));
#69485=CARTESIAN_POINT('Ctrl Pts',(-17.7432663110306,-17.0810404681722,
-16.9749607847386));
#69486=CARTESIAN_POINT('Ctrl Pts',(-17.7191978610519,-17.0940606039165,
-16.9766142811101));
#69487=CARTESIAN_POINT('Ctrl Pts',(-17.7116983322456,-17.0981765229141,
-16.9771295576006));
#69488=CARTESIAN_POINT('Ctrl Pts',(-17.6985890472135,-17.1054749523511,
-16.978030442223));
#69489=CARTESIAN_POINT('Ctrl Pts',(-17.6929685405135,-17.1086378287129,
-16.9784167463307));
#69490=CARTESIAN_POINT('Ctrl Pts',(-17.6820797469114,-17.1148310591907,
-16.9791652924963));
#69491=CARTESIAN_POINT('Ctrl Pts',(-17.6768098890246,-17.1178585097182,
-16.9795276341023));
#69492=CARTESIAN_POINT('Ctrl Pts',(-17.6642381533248,-17.1251529582114,
-16.9803922356098));
#69493=CARTESIAN_POINT('Ctrl Pts',(-17.6569486277487,-17.1294411210117,
-16.9808937250359));
#69494=CARTESIAN_POINT('Ctrl Pts',(-17.6307080097925,-17.1450899351325,
-16.9826997496359));
#69495=CARTESIAN_POINT('Ctrl Pts',(-17.6119089444366,-17.156703669194,-16.9839950615846));
#69496=CARTESIAN_POINT('Ctrl Pts',(-17.4368578876178,-17.268671144437,-16.996080703535));
#69497=CARTESIAN_POINT('Ctrl Pts',(-17.2942700190669,-17.388875794406,-17.0060131877644));
#69498=CARTESIAN_POINT('Ctrl Pts',(-17.1152583045133,-17.5853343146682,
-17.020502549017));
#69499=CARTESIAN_POINT('Ctrl Pts',(-17.0647361392392,-17.6475246522873,
-17.0249059401472));
#69500=CARTESIAN_POINT('Ctrl Pts',(-16.9967760617693,-17.7416121664945,
-17.0315450959902));
#69501=CARTESIAN_POINT('Ctrl Pts',(-16.9764405726915,-17.7713348355755,
-17.033639694912));
#69502=CARTESIAN_POINT('Ctrl Pts',(-16.9528175910555,-17.8078260828551,
-17.0362266564704));
#69503=CARTESIAN_POINT('Ctrl Pts',(-16.948794117962,-17.8141139417414,-17.0366729585263));
#69504=CARTESIAN_POINT('Ctrl Pts',(-16.9425809571116,-17.8239378959757,
-17.0373712988066));
#69505=CARTESIAN_POINT('Ctrl Pts',(-16.9403682463315,-17.8274594585754,
-17.0376218396951));
#69506=CARTESIAN_POINT('Ctrl Pts',(-16.9362776842916,-17.8340124367917,
-17.0380884819651));
#69507=CARTESIAN_POINT('Ctrl Pts',(-16.9343971097411,-17.8370420848076,
-17.0383043998584));
#69508=CARTESIAN_POINT('Ctrl Pts',(-16.9301549094423,-17.8439150585005,
-17.0387946140153));
#69509=CARTESIAN_POINT('Ctrl Pts',(-16.9277979197851,-17.8477611703697,
-17.0390692079335));
#69510=CARTESIAN_POINT('Ctrl Pts',(-16.9217434753202,-17.8577119995996,
-17.0397802858899));
#69511=CARTESIAN_POINT('Ctrl Pts',(-16.918064602519,-17.8638278776182,-17.0402179373027));
#69512=CARTESIAN_POINT('Ctrl Pts',(-16.8956519085938,-17.9015176509563,
-17.0429182214243));
#69513=CARTESIAN_POINT('Ctrl Pts',(-16.8777123346157,-17.9335538309219,
-17.0452271610942));
#69514=CARTESIAN_POINT('Ctrl Pts',(-16.7812822564166,-18.1167764476263,
-17.0584410732572));
#69515=CARTESIAN_POINT('Ctrl Pts',(-16.7204315137949,-18.2765372061968,
-17.0699344810719));
#69516=CARTESIAN_POINT('Ctrl Pts',(-16.6563721613909,-18.5345434963653,
-17.0872113786762));
#69517=CARTESIAN_POINT('Ctrl Pts',(-16.6396562682331,-18.628679777685,-17.0932786383464));
#69518=CARTESIAN_POINT('Ctrl Pts',(-16.6270442361961,-18.7449141568,-17.100460398315));
#69519=CARTESIAN_POINT('Ctrl Pts',(-16.6250581161765,-18.766227772416,-17.1017650734341));
#69520=CARTESIAN_POINT('Ctrl Pts',(-16.6226955460807,-18.7965531682359,
-17.1036046351112));
#69521=CARTESIAN_POINT('Ctrl Pts',(-16.6220529425179,-18.8055423441286,
-17.1041478411478));
#69522=CARTESIAN_POINT('Ctrl Pts',(-16.6210439472005,-18.8210484167295,
-17.1050813395013));
#69523=CARTESIAN_POINT('Ctrl Pts',(-16.6206502605931,-18.8275633548632,
-17.1054724834599));
#69524=CARTESIAN_POINT('Ctrl Pts',(-16.6199544879947,-18.8400350697693,
-17.1062192514445));
#69525=CARTESIAN_POINT('Ctrl Pts',(-16.6196474346163,-18.8459914965316,
-17.1065750276583));
#69526=CARTESIAN_POINT('Ctrl Pts',(-16.6189150607854,-18.8614706606631,
-17.1074973603473));
#69527=CARTESIAN_POINT('Ctrl Pts',(-16.6185288738891,-18.8709951823553,
-17.1080626861599));
#69528=CARTESIAN_POINT('Ctrl Pts',(-16.6174336371598,-18.90341491521,-17.1099797258332));
#69529=CARTESIAN_POINT('Ctrl Pts',(-16.6170318270614,-18.9263193886757,
-17.111321831094));
#69530=CARTESIAN_POINT('Ctrl Pts',(-16.616770440827,-19.1258378891143,-17.1229165409291));
#69531=CARTESIAN_POINT('Ctrl Pts',(-16.6386384415009,-19.30178164891,-17.1324069158117));
#69532=CARTESIAN_POINT('Ctrl Pts',(-16.7033227085838,-19.5565424655574,
-17.1467111447771));
#69533=CARTESIAN_POINT('Ctrl Pts',(-16.7296225909621,-19.6387246227305,
-17.1514333719584));
#69534=CARTESIAN_POINT('Ctrl Pts',(-16.774488171413,-19.7541333054791,-17.1585044308519));
#69535=CARTESIAN_POINT('Ctrl Pts',(-16.789051571883,-19.7888271415139,-17.1606901432653));
#69536=CARTESIAN_POINT('Ctrl Pts',(-16.8076413561941,-19.8300025809461,
-17.1633781442775));
#69537=CARTESIAN_POINT('Ctrl Pts',(-16.8107890970171,-19.8368762486663,
-17.1638300670417));
#69538=CARTESIAN_POINT('Ctrl Pts',(-16.8157341570418,-19.8475236603388,
-17.164535303506));
#69539=CARTESIAN_POINT('Ctrl Pts',(-16.8175059857057,-19.851309269922,-17.1647870716465));
#69540=CARTESIAN_POINT('Ctrl Pts',(-16.8208093596306,-19.8583130119818,
-17.1652548161795));
#69541=CARTESIAN_POINT('Ctrl Pts',(-16.8223378247949,-19.8615325334425,
-17.1654706015937));
#69542=CARTESIAN_POINT('Ctrl Pts',(-16.8258074231513,-19.8687934283163,
-17.1659589922363));
#69543=CARTESIAN_POINT('Ctrl Pts',(-16.8277532579283,-19.8728324809812,
-17.1662318856367));
#69544=CARTESIAN_POINT('Ctrl Pts',(-16.8335218106989,-19.8847098719027,
-17.1670378795736));
#69545=CARTESIAN_POINT('Ctrl Pts',(-16.8373800957909,-19.8925306938647,
-17.1675731172341));
#69546=CARTESIAN_POINT('Ctrl Pts',(-16.8651908430789,-19.9480366110126,
-17.1714028920744));
#69547=CARTESIAN_POINT('Ctrl Pts',(-16.8908884514517,-19.9948208753516,
-17.1747945565816));
#69548=CARTESIAN_POINT('Ctrl Pts',(-16.9273694294093,-20.0556686479437,
-17.1793797742828));
#69549=CARTESIAN_POINT('Ctrl Pts',(-16.9366033100326,-20.0706436509309,
-17.1805228082439));
#69550=CARTESIAN_POINT('Ctrl Pts',(-16.9719941498716,-20.126468915809,-17.1848347503723));
#69551=CARTESIAN_POINT('Ctrl Pts',(-16.9993654293923,-20.1665305753368,
-17.1880324235468));
#69552=CARTESIAN_POINT('Ctrl Pts',(-17.0928605092622,-20.2937580924798,
-17.1984619701991));
#69553=CARTESIAN_POINT('Ctrl Pts',(-17.1643723170991,-20.3767547191093,
-17.2056947721282));
#69554=CARTESIAN_POINT('Ctrl Pts',(-17.28107317332,-20.4926910179978,-17.2162684264486));
#69555=CARTESIAN_POINT('Ctrl Pts',(-17.3216672997978,-20.5299868002108,
-17.2197576559781));
#69556=CARTESIAN_POINT('Ctrl Pts',(-17.3898211222542,-20.5878633481733,
-17.2253153558215));
#69557=CARTESIAN_POINT('Ctrl Pts',(-17.4165057313679,-20.6094301848731,
-17.227422267129));
#69558=CARTESIAN_POINT('Ctrl Pts',(-17.4522728772119,-20.636927715525,-17.2301588454392));
#69559=CARTESIAN_POINT('Ctrl Pts',(-17.4608922188826,-20.6434497947852,
-17.2308118548246));
#69560=CARTESIAN_POINT('Ctrl Pts',(-17.4750937102978,-20.6540257155861,
-17.2318773604536));
#69561=CARTESIAN_POINT('Ctrl Pts',(-17.4806463151711,-20.6581187312863,
-17.2322913861736));
#69562=CARTESIAN_POINT('Ctrl Pts',(-17.491434844316,-20.6659902342917,-17.2330909019716));
#69563=CARTESIAN_POINT('Ctrl Pts',(-17.4966682378424,-20.6697720457467,
-17.2334765184006));
#69564=CARTESIAN_POINT('Ctrl Pts',(-17.508794110066,-20.6784504068582,-17.2343649355882));
#69565=CARTESIAN_POINT('Ctrl Pts',(-17.5156988128512,-20.6833297492462,
-17.2348670702967));
#69566=CARTESIAN_POINT('Ctrl Pts',(-17.5343516583174,-20.6963443035617,
-17.2362136679501));
#69567=CARTESIAN_POINT('Ctrl Pts',(-17.5461533725958,-20.7044022362873,
-17.2370551895728));
#69568=CARTESIAN_POINT('Ctrl Pts',(-17.6551775605434,-20.7772339086621,
-17.2447362506206));
#69569=CARTESIAN_POINT('Ctrl Pts',(-17.7575296766802,-20.8339797147863,
-17.2512591827382));
#69570=CARTESIAN_POINT('Ctrl Pts',(-18.0124219919546,-20.9488725005736,
-17.2665652530841));
#69571=CARTESIAN_POINT('Ctrl Pts',(-18.1679882457019,-20.9984098918762,
-17.2751653043777));
#69572=CARTESIAN_POINT('Ctrl Pts',(-18.3595750826726,-21.0358790289379,
-17.2863743156676));
#69573=CARTESIAN_POINT('Ctrl Pts',(-18.3916170567969,-21.0413825606828,
-17.288270383163));
#69574=CARTESIAN_POINT('Ctrl Pts',(-18.4309324842728,-21.0472067901356,
-17.2906368068298));
#69575=CARTESIAN_POINT('Ctrl Pts',(-18.4380992549803,-21.0482309410399,
-17.2910697957271));
#69576=CARTESIAN_POINT('Ctrl Pts',(-18.4493423236919,-21.0497788007801,
-17.2917517878829));
#69577=CARTESIAN_POINT('Ctrl Pts',(-18.4534152114387,-21.0503274447643,
-17.2919994053521));
#69578=CARTESIAN_POINT('Ctrl Pts',(-18.4610309745763,-21.0513307671587,
-17.2924635078914));
#69579=CARTESIAN_POINT('Ctrl Pts',(-18.4645734119163,-21.0517883397518,
-17.2926798275905));
#69580=CARTESIAN_POINT('Ctrl Pts',(-18.4726622072493,-21.0528123543676,
-17.2931747771159));
#69581=CARTESIAN_POINT('Ctrl Pts',(-18.4772092407399,-21.0533730024036,
-17.293453728814));
#69582=CARTESIAN_POINT('Ctrl Pts',(-18.4911905548546,-21.0550508380933,
-17.2943135949957));
#69583=CARTESIAN_POINT('Ctrl Pts',(-18.5006304132317,-21.0561192652739,
-17.2948971486615));
#69584=CARTESIAN_POINT('Ctrl Pts',(-18.5854810223028,-21.0651448653258,
-17.3001673611239));
#69585=CARTESIAN_POINT('Ctrl Pts',(-18.6612537132996,-21.0691075897821,
-17.3050487058846));
#69586=CARTESIAN_POINT('Ctrl Pts',(-18.9219965594145,-21.0687299178882,
-17.3221015383477));
#69587=CARTESIAN_POINT('Ctrl Pts',(-19.1061342193762,-21.0442294878566,
-17.3344988871995));
#69588=CARTESIAN_POINT('Ctrl Pts',(-19.3361763460763,-20.9822486172945,
-17.3495263661884));
#69589=CARTESIAN_POINT('Ctrl Pts',(-19.3870659874507,-20.9664556124278,
-17.3528279537341));
#69590=CARTESIAN_POINT('Ctrl Pts',(-19.449137866429,-20.9445923063702,-17.3568296339874));
#69591=CARTESIAN_POINT('Ctrl Pts',(-19.4609291538828,-20.9403209708827,
-17.3575886868804));
#69592=CARTESIAN_POINT('Ctrl Pts',(-19.4795054214978,-20.9334044716238,
-17.3587829174995));
#69593=CARTESIAN_POINT('Ctrl Pts',(-19.4863157631402,-20.930828696034,-17.3592203989941));
#69594=CARTESIAN_POINT('Ctrl Pts',(-19.4990578944801,-20.9259341372074,
-17.3600383309089));
#69595=CARTESIAN_POINT('Ctrl Pts',(-19.5049927555579,-20.9236236284308,
-17.360419053224));
#69596=CARTESIAN_POINT('Ctrl Pts',(-19.5182499787068,-20.9183934271379,
-17.3612690029372));
#69597=CARTESIAN_POINT('Ctrl Pts',(-19.5255666661395,-20.9154595374035,
-17.3617377465269));
#69598=CARTESIAN_POINT('Ctrl Pts',(-19.5440619417602,-20.9079230021293,
-17.3629218690996));
#69599=CARTESIAN_POINT('Ctrl Pts',(-19.5552179008716,-20.9032653095175,
-17.3636353825342));
#69600=CARTESIAN_POINT('Ctrl Pts',(-19.6186384189793,-20.876146536511,-17.3676884087989));
#69601=CARTESIAN_POINT('Ctrl Pts',(-19.6700234558743,-20.8516804855319,
-17.3709588146022));
#69602=CARTESIAN_POINT('Ctrl Pts',(-19.744123272148,-20.8126614410897,-17.3756896257241));
#69603=CARTESIAN_POINT('Ctrl Pts',(-19.7676428155683,-20.7996992781501,
-17.3771936400324));
#69604=CARTESIAN_POINT('Ctrl Pts',(-19.8912853531918,-20.7284570932604,
-17.3851311464127));
#69605=CARTESIAN_POINT('Ctrl Pts',(-19.9867437427206,-20.662480368478,-17.3913560778331));
#69606=CARTESIAN_POINT('Ctrl Pts',(-20.1382166992282,-20.5382755794598,
-17.4020349591394));
#69607=CARTESIAN_POINT('Ctrl Pts',(-20.1971741751657,-20.4840620368269,
-17.406436719338));
#69608=CARTESIAN_POINT('Ctrl Pts',(-20.277994110509,-20.4008158256283,-17.4130736571843));
#69609=CARTESIAN_POINT('Ctrl Pts',(-20.3024071722651,-20.3743514699397,
-17.4151677775558));
#69610=CARTESIAN_POINT('Ctrl Pts',(-20.3310517304236,-20.3416656034103,
-17.4177542081874));
#69611=CARTESIAN_POINT('Ctrl Pts',(-20.3359416575026,-20.3360258816741,
-17.418200479953));
#69612=CARTESIAN_POINT('Ctrl Pts',(-20.3435094272081,-20.3272038759969,
-17.4188987830594));
#69613=CARTESIAN_POINT('Ctrl Pts',(-20.3462079462934,-20.3240392975618,
-17.4191493173223));
#69614=CARTESIAN_POINT('Ctrl Pts',(-20.3512028609173,-20.318146632908,-17.4196159536965));
#69615=CARTESIAN_POINT('Ctrl Pts',(-20.3535016950404,-20.3154206889733,
-17.4198318723601));
#69616=CARTESIAN_POINT('Ctrl Pts',(-20.3586930877582,-20.3092331119848,
-17.4203220966116));
#69617=CARTESIAN_POINT('Ctrl Pts',(-20.3615814610908,-20.305768051152,-17.4205966999062));
#69618=CARTESIAN_POINT('Ctrl Pts',(-20.3701034798719,-20.2954778465404,
-17.4214123466882));
#69619=CARTESIAN_POINT('Ctrl Pts',(-20.3757053452268,-20.288626677189,-17.4219556028854));
#69620=CARTESIAN_POINT('Ctrl Pts',(-20.4168973094689,-20.2375986553026,
-17.4260020148012));
#69621=CARTESIAN_POINT('Ctrl Pts',(-20.4507386861598,-20.1920460965375,
-17.4296148682213));
#69622=CARTESIAN_POINT('Ctrl Pts',(-20.517596219775,-20.0940618788603,-17.4372975613278));
#69623=CARTESIAN_POINT('Ctrl Pts',(-20.5502247308369,-20.0414255110625,
-17.4413751905982));
#69624=CARTESIAN_POINT('Ctrl Pts',(-20.6341054112911,-19.891840852066,-17.4527033103477));
#69625=CARTESIAN_POINT('Ctrl Pts',(-20.6802113289033,-19.7922180217654,
-17.4599518896997));
#69626=CARTESIAN_POINT('Ctrl Pts',(-20.7198023112215,-19.6856855302226,
-17.4672586538775));
#69627=CARTESIAN_POINT('Ctrl Pts',(-20.7211968761186,-19.6818998908439,
-17.467517754415));
#69628=CARTESIAN_POINT('Ctrl Pts',(-20.7225805818549,-19.6781103700332,
-17.4677765722177));
#69629=CARTESIAN_POINT('',(-20.8509993557814,-18.9503484488822,-16.4878149381751));
#69630=CARTESIAN_POINT('Ctrl Pts',(-20.7225805822089,-19.6781103690637,
-17.242699000807));
#69631=CARTESIAN_POINT('Ctrl Pts',(-20.7071866862069,-19.7202692528619,
-17.2398827936462));
#69632=CARTESIAN_POINT('Ctrl Pts',(-20.690454937598,-19.7619308775447,-17.2371085597985));
#69633=CARTESIAN_POINT('Ctrl Pts',(-20.6673796263601,-19.8144898843245,
-17.2336175936552));
#69634=CARTESIAN_POINT('Ctrl Pts',(-20.6622477609682,-19.8259028338721,
-17.2328600682927));
#69635=CARTESIAN_POINT('Ctrl Pts',(-20.6539422314611,-19.8439444038136,
-17.2316632398376));
#69636=CARTESIAN_POINT('Ctrl Pts',(-20.6508347871509,-19.8506030227701,
-17.231221670051));
#69637=CARTESIAN_POINT('Ctrl Pts',(-20.6449719417752,-19.8629971034382,
-17.2303999732908));
#69638=CARTESIAN_POINT('Ctrl Pts',(-20.642225237177,-19.8687365653734,-17.2300195510647));
#69639=CARTESIAN_POINT('Ctrl Pts',(-20.6360566856785,-19.8814784045976,
-17.2291751572373));
#69640=CARTESIAN_POINT('Ctrl Pts',(-20.6326219514571,-19.8884744673926,
-17.2287116400382));
#69641=CARTESIAN_POINT('Ctrl Pts',(-20.6224963090696,-19.9088142493045,
-17.2273642520349));
#69642=CARTESIAN_POINT('Ctrl Pts',(-20.6157027234671,-19.9221065377609,
-17.2264839788105));
#69643=CARTESIAN_POINT('Ctrl Pts',(-20.5587597245865,-20.0306717084962,
-17.2192939450419));
#69644=CARTESIAN_POINT('Ctrl Pts',(-20.5015468824836,-20.1220697236977,
-17.2132499861037));
#69645=CARTESIAN_POINT('Ctrl Pts',(-20.358246833973,-20.316327360521,-17.1999842110649));
#69646=CARTESIAN_POINT('Ctrl Pts',(-20.2688620494572,-20.4161593055845,
-17.1928654177092));
#69647=CARTESIAN_POINT('Ctrl Pts',(-20.1586099418722,-20.5180283742549,
-17.1845194666834));
#69648=CARTESIAN_POINT('Ctrl Pts',(-20.1464267508641,-20.5290253673553,
-17.1836022384472));
#69649=CARTESIAN_POINT('Ctrl Pts',(-20.0943129960234,-20.5749768186359,
-17.1796939028036));
#69650=CARTESIAN_POINT('Ctrl Pts',(-20.0532066678058,-20.6085620917094,
-17.1766481849095));
#69651=CARTESIAN_POINT('Ctrl Pts',(-20.0039435205832,-20.6458146936984,
-17.1729828937423));
#69652=CARTESIAN_POINT('Ctrl Pts',(-19.9969687336073,-20.6510216991269,
-17.1724636086201));
#69653=CARTESIAN_POINT('Ctrl Pts',(-19.9863559594371,-20.6588431735676,
-17.1716726166858));
#69654=CARTESIAN_POINT('Ctrl Pts',(-19.9827413591033,-20.6614894224618,
-17.1714030646887));
#69655=CARTESIAN_POINT('Ctrl Pts',(-19.9762362410141,-20.6662201789241,
-17.1709176382968));
#69656=CARTESIAN_POINT('Ctrl Pts',(-19.9733488372088,-20.6683088765515,
-17.1707020588194));
#69657=CARTESIAN_POINT('Ctrl Pts',(-19.967061127155,-20.6728331558745,-17.1702323444344));
#69658=CARTESIAN_POINT('Ctrl Pts',(-19.9636589172788,-20.6752659226353,
-17.1699780273047));
#69659=CARTESIAN_POINT('Ctrl Pts',(-19.954076393472,-20.6820751266686,-17.1692613320313));
#69660=CARTESIAN_POINT('Ctrl Pts',(-19.9478798457932,-20.6864284550889,
-17.1687974193406));
#69661=CARTESIAN_POINT('Ctrl Pts',(-19.9105768638137,-20.712337509496,-17.1660025855319));
#69662=CARTESIAN_POINT('Ctrl Pts',(-19.87892237179,-20.7330877619598,-17.1636223318261));
#69663=CARTESIAN_POINT('Ctrl Pts',(-19.7726421312894,-20.7987528646892,
-17.1556460148323));
#69664=CARTESIAN_POINT('Ctrl Pts',(-19.6958035077543,-20.839910409374,-17.1499068520919));
#69665=CARTESIAN_POINT('Ctrl Pts',(-19.4572948563072,-20.9493163566282,
-17.1325694314782));
#69666=CARTESIAN_POINT('Ctrl Pts',(-19.2894380187928,-21.0023512103457,
-17.1210591786638));
#69667=CARTESIAN_POINT('Ctrl Pts',(-19.0943178486237,-21.0382380192877,
-17.1088476171765));
#69668=CARTESIAN_POINT('Ctrl Pts',(-19.0716297582314,-21.0420297215623,
-17.1074435045073));
#69669=CARTESIAN_POINT('Ctrl Pts',(-19.0394421739339,-21.0468711742535,
-17.1054731158105));
#69670=CARTESIAN_POINT('Ctrl Pts',(-19.0299910750183,-21.0482274319636,
-17.1048971817548));
#69671=CARTESIAN_POINT('Ctrl Pts',(-19.01461882742,-21.0503273528613,-17.1039645972939));
#69672=CARTESIAN_POINT('Ctrl Pts',(-19.008703218845,-21.051109989676,-17.103606718715));
#69673=CARTESIAN_POINT('Ctrl Pts',(-18.996312872,-21.0526959616169,-17.1028592026194));
#69674=CARTESIAN_POINT('Ctrl Pts',(-18.989837561471,-21.0534943991314,-17.1024697234617));
#69675=CARTESIAN_POINT('Ctrl Pts',(-18.9744229206164,-21.0553227971764,
-17.1015453145216));
#69676=CARTESIAN_POINT('Ctrl Pts',(-18.9654804646222,-21.0563257276822,
-17.1010112420568));
#69677=CARTESIAN_POINT('Ctrl Pts',(-18.935326154409,-21.059513103711,-17.0992175417359));
#69678=CARTESIAN_POINT('Ctrl Pts',(-18.9140873320884,-21.0614341194959,
-17.0979661977834));
#69679=CARTESIAN_POINT('Ctrl Pts',(-18.7982699741764,-21.0701475770386,
-17.0912026408854));
#69680=CARTESIAN_POINT('Ctrl Pts',(-18.7033405889997,-21.070901323857,-17.0858836269407));
#69681=CARTESIAN_POINT('Ctrl Pts',(-18.4394889542103,-21.0552535595164,
-17.071340366986));
#69682=CARTESIAN_POINT('Ctrl Pts',(-18.2721439774644,-21.0249423035023,
-17.0624221720012));
#69683=CARTESIAN_POINT('Ctrl Pts',(-18.0737080529918,-20.9637563220821,
-17.0505790012312));
#69684=CARTESIAN_POINT('Ctrl Pts',(-18.0375090321643,-20.9515121601701,
-17.0483619499862));
#69685=CARTESIAN_POINT('Ctrl Pts',(-17.9948825451487,-20.9357960135558,
-17.0456614960739));
#69686=CARTESIAN_POINT('Ctrl Pts',(-17.9881143132747,-20.9332611575503,
-17.0452299896042));
#69687=CARTESIAN_POINT('Ctrl Pts',(-17.9771174268945,-20.9290782400852,
-17.0445242321988));
#69688=CARTESIAN_POINT('Ctrl Pts',(-17.9728807944107,-20.9274511259182,
-17.0442512042675));
#69689=CARTESIAN_POINT('Ctrl Pts',(-17.9653227269763,-20.9245204640644,
-17.043762052238));
#69690=CARTESIAN_POINT('Ctrl Pts',(-17.9619993258327,-20.9232221310761,
-17.0435462428319));
#69691=CARTESIAN_POINT('Ctrl Pts',(-17.9548275239862,-20.9203994477586,
-17.0430789581784));
#69692=CARTESIAN_POINT('Ctrl Pts',(-17.9509803611275,-20.9188722321941,
-17.0428273165514));
#69693=CARTESIAN_POINT('Ctrl Pts',(-17.9402917488547,-20.9145928238902,
-17.0421255088));
#69694=CARTESIAN_POINT('Ctrl Pts',(-17.9334602411006,-20.9118161829777,
-17.0416739067873));
#69695=CARTESIAN_POINT('Ctrl Pts',(-17.8947048219833,-20.8958277432965,
-17.039095154228));
#69696=CARTESIAN_POINT('Ctrl Pts',(-17.8630955614699,-20.8818724911,-17.0369269617804));
#69697=CARTESIAN_POINT('Ctrl Pts',(-17.7641898542309,-20.83528171978,-17.0299668299418));
#69698=CARTESIAN_POINT('Ctrl Pts',(-17.6982762974552,-20.7998518963342,
-17.0250666955627));
#69699=CARTESIAN_POINT('Ctrl Pts',(-17.4686460672905,-20.6602696858083,
-17.0073424438745));
#69700=CARTESIAN_POINT('Ctrl Pts',(-17.3175009378047,-20.5372027735794,
-16.994526052063));
#69701=CARTESIAN_POINT('Ctrl Pts',(-17.1708028446326,-20.3797783180298,
-16.9813057681638));
#69702=CARTESIAN_POINT('Ctrl Pts',(-17.1566170577805,-20.364090427883,-16.9800162855291));
#69703=CARTESIAN_POINT('Ctrl Pts',(-17.137192247565,-20.3419506986549,-16.9782343438223));
#69704=CARTESIAN_POINT('Ctrl Pts',(-17.1317528823488,-20.3356770287819,
-16.9777335321091));
#69705=CARTESIAN_POINT('Ctrl Pts',(-17.1224225354394,-20.3247867729303,
-16.9768712312965));
#69706=CARTESIAN_POINT('Ctrl Pts',(-17.1185141624667,-20.3201852791619,
-16.9765090250333));
#69707=CARTESIAN_POINT('Ctrl Pts',(-17.1104566484757,-20.3106161623903,
-16.9757601894134));
#69708=CARTESIAN_POINT('Ctrl Pts',(-17.1063104930697,-20.3056460990419,
-16.9753736847491));
#69709=CARTESIAN_POINT('Ctrl Pts',(-17.0966453061623,-20.2939516686291,
-16.9744698764629));
#69710=CARTESIAN_POINT('Ctrl Pts',(-17.0911447734072,-20.2872121113402,
-16.9739533276104));
#69711=CARTESIAN_POINT('Ctrl Pts',(-17.0733833441665,-20.2651738996425,
-16.9722780336536));
#69712=CARTESIAN_POINT('Ctrl Pts',(-17.061293164061,-20.2497385127684,-16.9711261320998));
#69713=CARTESIAN_POINT('Ctrl Pts',(-17.0003348531068,-20.1696462749427,
-16.9652542428423));
#69714=CARTESIAN_POINT('Ctrl Pts',(-16.9549916123088,-20.1023862495792,
-16.960673051698));
#69715=CARTESIAN_POINT('Ctrl Pts',(-16.8275352258754,-19.8876892612267,
-16.9468346645544));
#69716=CARTESIAN_POINT('Ctrl Pts',(-16.7590966086046,-19.732942507968,-16.9379622994223));
#69717=CARTESIAN_POINT('Ctrl Pts',(-16.693950348518,-19.5201514423581,-16.9254531481011));
#69718=CARTESIAN_POINT('Ctrl Pts',(-16.6801381357566,-19.4679932502747,
-16.9223592526132));
#69719=CARTESIAN_POINT('Ctrl Pts',(-16.6664201032264,-19.4068393105263,
-16.9186401764896));
#69720=CARTESIAN_POINT('Ctrl Pts',(-16.6645594797102,-19.3982973839974,
-16.9181186432813));
#69721=CARTESIAN_POINT('Ctrl Pts',(-16.661823846647,-19.3853533563472,-16.9173248934283));
#69722=CARTESIAN_POINT('Ctrl Pts',(-16.6609098159649,-19.3809594735953,
-16.917054854149));
#69723=CARTESIAN_POINT('Ctrl Pts',(-16.6592949574965,-19.3730708857045,
-16.9165689095406));
#69724=CARTESIAN_POINT('Ctrl Pts',(-16.6585889778861,-19.3695772900585,
-16.9163533019061));
#69725=CARTESIAN_POINT('Ctrl Pts',(-16.6570749505426,-19.3619863167144,
-16.9158839466009));
#69726=CARTESIAN_POINT('Ctrl Pts',(-16.6562702140935,-19.3578883799985,
-16.9156300190016));
#69727=CARTESIAN_POINT('Ctrl Pts',(-16.6540458423031,-19.3463813039791,
-16.9149154975508));
#69728=CARTESIAN_POINT('Ctrl Pts',(-16.6526536943265,-19.3389670050186,
-16.9144533837424));
#69729=CARTESIAN_POINT('Ctrl Pts',(-16.6446066028301,-19.2948098084948,
-16.9116915464598));
#69730=CARTESIAN_POINT('Ctrl Pts',(-16.6388855588433,-19.2579058937774,
-16.9093438074189));
#69731=CARTESIAN_POINT('Ctrl Pts',(-16.6233337069865,-19.1364482469166,
-16.9015292338294));
#69732=CARTESIAN_POINT('Ctrl Pts',(-16.6176256454316,-19.051453917579,-16.8959251206881));
#69733=CARTESIAN_POINT('Ctrl Pts',(-16.6158406826574,-18.78818729055,-16.878533024447));
#69734=CARTESIAN_POINT('Ctrl Pts',(-16.6371296155216,-18.6105434024813,
-16.8668240609378));
#69735=CARTESIAN_POINT('Ctrl Pts',(-16.6859698298717,-18.4155483783197,
-16.8544535671671));
#69736=CARTESIAN_POINT('Ctrl Pts',(-16.6918609646271,-18.3935412781592,
-16.8530631262047));
#69737=CARTESIAN_POINT('Ctrl Pts',(-16.7007138570992,-18.362485854435,-16.8511084190362));
#69738=CARTESIAN_POINT('Ctrl Pts',(-16.7033830170029,-18.3533564167923,
-16.8505347020114));
#69739=CARTESIAN_POINT('Ctrl Pts',(-16.7078248126257,-18.3385355447495,
-16.8496047265275));
#69740=CARTESIAN_POINT('Ctrl Pts',(-16.7095600960045,-18.3328331371699,
-16.8492472534786));
#69741=CARTESIAN_POINT('Ctrl Pts',(-16.7132468937457,-18.3208989578979,
-16.8484998057258));
#69742=CARTESIAN_POINT('Ctrl Pts',(-16.7152032074452,-18.314668725369,-16.8481099928008));
#69743=CARTESIAN_POINT('Ctrl Pts',(-16.7199334445207,-18.2998447620535,
-16.8471833733078));
#69744=CARTESIAN_POINT('Ctrl Pts',(-16.7227336023176,-18.2912594868768,
-16.846647435122));
#69745=CARTESIAN_POINT('Ctrl Pts',(-16.7323900265568,-18.2622831702968,
-16.8448407869392));
#69746=CARTESIAN_POINT('Ctrl Pts',(-16.7395022823547,-18.2419783838035,
-16.8435785272793));
#69747=CARTESIAN_POINT('Ctrl Pts',(-16.8090401333256,-18.0527504743123,
-16.8318408310221));
#69748=CARTESIAN_POINT('Ctrl Pts',(-16.8924688536244,-17.8923348809369,
-16.8221685232437));
#69749=CARTESIAN_POINT('Ctrl Pts',(-17.0635436363908,-17.6460073937686,
-16.8058446646909));
#69750=CARTESIAN_POINT('Ctrl Pts',(-17.1401008123895,-17.5536015661253,
-16.7992692549738));
#69751=CARTESIAN_POINT('Ctrl Pts',(-17.230717692082,-17.4613887419886,-16.7916073449943));
#69752=CARTESIAN_POINT('Ctrl Pts',(-17.2374355232953,-17.454644204198,-16.7910399395474));
#69753=CARTESIAN_POINT('Ctrl Pts',(-17.2474561487413,-17.4447185388798,
-16.790194038014));
#69754=CARTESIAN_POINT('Ctrl Pts',(-17.25072426686,-17.4415023590478,-16.7899182289783));
#69755=CARTESIAN_POINT('Ctrl Pts',(-17.2565570365676,-17.4357994687324,
-16.7894260507636));
#69756=CARTESIAN_POINT('Ctrl Pts',(-17.2591175591865,-17.4333086071344,
-16.789210012053));
#69757=CARTESIAN_POINT('Ctrl Pts',(-17.2646356565874,-17.4279677511664,
-16.7887444657326));
#69758=CARTESIAN_POINT('Ctrl Pts',(-17.2675951807656,-17.4251199213295,
-16.7884948036104));
#69759=CARTESIAN_POINT('Ctrl Pts',(-17.2757860291863,-17.4172839794755,
-16.7878039492048));
#69760=CARTESIAN_POINT('Ctrl Pts',(-17.281034585023,-17.4123140749686,-16.7873613917444));
#69761=CARTESIAN_POINT('Ctrl Pts',(-17.3099070969077,-17.3852535322104,
-16.7849280974778));
#69762=CARTESIAN_POINT('Ctrl Pts',(-17.3340081094426,-17.3636809096826,
-16.782901456387));
#69763=CARTESIAN_POINT('Ctrl Pts',(-17.4824025498713,-17.236856144322,-16.7704995961213));
#69764=CARTESIAN_POINT('Ctrl Pts',(-17.6180060813219,-17.1456854922775,
-16.7595313373077));
#69765=CARTESIAN_POINT('Ctrl Pts',(-17.8665964558168,-17.0173249683642,
-16.7412563215257));
#69766=CARTESIAN_POINT('Ctrl Pts',(-17.9747506811773,-16.9723776410568,
-16.7338093065157));
#69767=CARTESIAN_POINT('Ctrl Pts',(-18.0996607031708,-16.9322212624601,
-16.725798119577));
#69768=CARTESIAN_POINT('Ctrl Pts',(-18.1132852745798,-16.9279926538168,
-16.7249316381733));
#69769=CARTESIAN_POINT('Ctrl Pts',(-18.1350445415138,-16.9214796926512,
-16.7235592414817));
#69770=CARTESIAN_POINT('Ctrl Pts',(-18.1431517848276,-16.9191058193637,
-16.7230504107868));
#69771=CARTESIAN_POINT('Ctrl Pts',(-18.1574792978406,-16.9150035458274,
-16.722155532609));
#69772=CARTESIAN_POINT('Ctrl Pts',(-18.1636936307481,-16.9132549642114,
-16.7217688313049));
#69773=CARTESIAN_POINT('Ctrl Pts',(-18.1765673585127,-16.9096960380549,
-16.7209706665603));
#69774=CARTESIAN_POINT('Ctrl Pts',(-18.1832278091489,-16.9078897734488,
-16.7205593397101));
#69775=CARTESIAN_POINT('Ctrl Pts',(-18.2003552145358,-16.9033347388086,
-16.7195056937699));
#69776=CARTESIAN_POINT('Ctrl Pts',(-18.2108347110444,-16.9006335782022,
-16.7188649213668));
#69777=CARTESIAN_POINT('Ctrl Pts',(-18.2547291176205,-16.889677743759,-16.7161968238502));
#69778=CARTESIAN_POINT('Ctrl Pts',(-18.2883232148034,-16.8821579603937,
-16.7141931955809));
#69779=CARTESIAN_POINT('Ctrl Pts',(-18.3763862066593,-16.8646893451843,
-16.7090285773441));
#69780=CARTESIAN_POINT('Ctrl Pts',(-18.4310892375177,-16.8560517378061,
-16.7059073901907));
#69781=CARTESIAN_POINT('Ctrl Pts',(-18.5948725391548,-16.8367376252915,
-16.6967392121255));
#69782=CARTESIAN_POINT('Ctrl Pts',(-18.7045087158893,-16.832372087458,-16.690840869258));
#69783=CARTESIAN_POINT('Ctrl Pts',(-18.8740567160749,-16.8387829452223,
-16.6816022197807));
#69784=CARTESIAN_POINT('Ctrl Pts',(-18.9339971675003,-16.8436113513292,
-16.6783108407253));
#69785=CARTESIAN_POINT('Ctrl Pts',(-19.0516894609793,-16.8581560058829,
-16.6716691057979));
#69786=CARTESIAN_POINT('Ctrl Pts',(-19.1094034033004,-16.8677302851486,
-16.6683254482368));
#69787=CARTESIAN_POINT('Ctrl Pts',(-19.1753664736535,-16.8815014889161,
-16.6643281468837));
#69788=CARTESIAN_POINT('Ctrl Pts',(-19.1840799764115,-16.8833781261451,
-16.6637965388849));
#69789=CARTESIAN_POINT('Ctrl Pts',(-19.1971982837832,-16.8862902377051,
-16.6629904394672));
#69790=CARTESIAN_POINT('Ctrl Pts',(-19.2016121709663,-16.8872849279304,
-16.6627182278152));
#69791=CARTESIAN_POINT('Ctrl Pts',(-19.2094999626009,-16.8890890690967,
-16.662229956609));
#69792=CARTESIAN_POINT('Ctrl Pts',(-19.2129750399456,-16.8898931564741,
-16.6620142071101));
#69793=CARTESIAN_POINT('Ctrl Pts',(-19.2204880050938,-16.8916515742056,
-16.6615463786556));
#69794=CARTESIAN_POINT('Ctrl Pts',(-19.224525068488,-16.8926089804809,-16.6612941297055));
#69795=CARTESIAN_POINT('Ctrl Pts',(-19.2357732147725,-16.8953114756195,
-16.6605889512874));
#69796=CARTESIAN_POINT('Ctrl Pts',(-19.2429778949755,-16.8970825943458,
-16.6601345638521));
#69797=CARTESIAN_POINT('Ctrl Pts',(-19.2843731053505,-16.9074897841288,
-16.6575088449693));
#69798=CARTESIAN_POINT('Ctrl Pts',(-19.3183507857377,-16.9169406888622,
-16.6552947366187));
#69799=CARTESIAN_POINT('Ctrl Pts',(-19.4260418951529,-16.9498141803089,
-16.6481220216415));
#69800=CARTESIAN_POINT('Ctrl Pts',(-19.4987119360344,-16.9764281657833,
-16.6430482549039));
#69801=CARTESIAN_POINT('Ctrl Pts',(-19.7400456206873,-17.0801257844027,
-16.6257144912326));
#69802=CARTESIAN_POINT('Ctrl Pts',(-19.9000262360672,-17.1753597451589,
-16.6134772632227));
#69803=CARTESIAN_POINT('Ctrl Pts',(-20.065107849679,-17.3056524096765,-16.6005085396931));
#69804=CARTESIAN_POINT('Ctrl Pts',(-20.0843724871826,-17.3214164466501,
-16.5989872567154));
#69805=CARTESIAN_POINT('Ctrl Pts',(-20.1108795009821,-17.3438988898489,
-16.5968820931309));
#69806=CARTESIAN_POINT('Ctrl Pts',(-20.1183590845592,-17.3503332834673,
-16.5962866999898));
#69807=CARTESIAN_POINT('Ctrl Pts',(-20.1303340992737,-17.3607814748257,
-16.5953311476197));
#69808=CARTESIAN_POINT('Ctrl Pts',(-20.1348577854917,-17.3647625326856,
-16.5949696389318));
#69809=CARTESIAN_POINT('Ctrl Pts',(-20.1439190803303,-17.3728058140691,
-16.5942443919374));
#69810=CARTESIAN_POINT('Ctrl Pts',(-20.1484562811448,-17.3768684118831,
-16.5938806743387));
#69811=CARTESIAN_POINT('Ctrl Pts',(-20.1591620619209,-17.3865379008501,
-16.5930210682899));
#69812=CARTESIAN_POINT('Ctrl Pts',(-20.165315210729,-17.3921617849334,-16.5925259031136));
#69813=CARTESIAN_POINT('Ctrl Pts',(-20.184442593567,-17.4098524028828,-16.5909830312592));
#69814=CARTESIAN_POINT('Ctrl Pts',(-20.1972988745386,-17.4220459612747,
-16.5899407438504));
#69815=CARTESIAN_POINT('Ctrl Pts',(-20.2268685762946,-17.4508051194123,
-16.5875298221538));
#69816=CARTESIAN_POINT('Ctrl Pts',(-20.2434620592698,-17.4674909870972,
-16.5861664509592));
#69817=CARTESIAN_POINT('Ctrl Pts',(-20.2997786791785,-17.5260419643163,
-16.5814972966395));
#69818=CARTESIAN_POINT('Ctrl Pts',(-20.3380674688943,-17.569253648664,-16.5782491676903));
#69819=CARTESIAN_POINT('Ctrl Pts',(-20.4763746941787,-17.738831802744,-16.5661065345472));
#69820=CARTESIAN_POINT('Ctrl Pts',(-20.5636115001708,-17.8748912568406,
-16.5576023127839));
#69821=CARTESIAN_POINT('Ctrl Pts',(-20.6416459971465,-18.0339402135876,
-16.5477154509039));
#69822=CARTESIAN_POINT('Ctrl Pts',(-20.6485568417914,-18.0484408698823,
-16.5468141071445));
#69823=CARTESIAN_POINT('Ctrl Pts',(-20.6755174583762,-18.1067092160545,
-16.5431871370101));
#69824=CARTESIAN_POINT('Ctrl Pts',(-20.6942352162063,-18.1510732387471,
-16.5404143891016));
#69825=CARTESIAN_POINT('Ctrl Pts',(-20.7141874622809,-18.2032633720555,
-16.5370970994278));
#69826=CARTESIAN_POINT('Ctrl Pts',(-20.7169120126994,-18.210509022611,-16.5366353337055));
#69827=CARTESIAN_POINT('Ctrl Pts',(-20.72120687568,-18.2221237183024,-16.5358929335549));
#69828=CARTESIAN_POINT('Ctrl Pts',(-20.7228026895865,-18.2264833466497,
-16.5356137777783));
#69829=CARTESIAN_POINT('Ctrl Pts',(-20.7256062610715,-18.2342212233973,
-16.5351173748902));
#69830=CARTESIAN_POINT('Ctrl Pts',(-20.7268197865733,-18.2375973338817,
-16.5349004746183));
#69831=CARTESIAN_POINT('Ctrl Pts',(-20.729376641007,-18.2447678865605,-16.5344391096293));
#69832=CARTESIAN_POINT('Ctrl Pts',(-20.7307177109276,-18.248563020591,-16.5341945215084));
#69833=CARTESIAN_POINT('Ctrl Pts',(-20.7343141464232,-18.2588338316283,
-16.5335315464735));
#69834=CARTESIAN_POINT('Ctrl Pts',(-20.7365488624792,-18.2653166146142,
-16.5331119673121));
#69835=CARTESIAN_POINT('Ctrl Pts',(-20.7475603537765,-18.2977712382975,
-16.5310062601364));
#69836=CARTESIAN_POINT('Ctrl Pts',(-20.755863102756,-18.3238996905106,-16.529294496797));
#69837=CARTESIAN_POINT('Ctrl Pts',(-20.7784982102654,-18.4002373205132,
-16.524260424197));
#69838=CARTESIAN_POINT('Ctrl Pts',(-20.7914828668915,-18.4508228823952,
-16.5208839991854));
#69839=CARTESIAN_POINT('Ctrl Pts',(-20.8346493259577,-18.6491790801985,
-16.5076111963695));
#69840=CARTESIAN_POINT('Ctrl Pts',(-20.8508817057974,-18.7995417691991,
-16.4975179105289));
#69841=CARTESIAN_POINT('Ctrl Pts',(-20.8509993557814,-18.9503484488822,
-16.4878149381751));
#69842=CARTESIAN_POINT('Ctrl Pts',(-20.8509993578169,-18.9503510600803,
-16.4878147701694));
#69843=CARTESIAN_POINT('Ctrl Pts',(-20.8510649773497,-19.0345970093956,
-16.4823943487751));
#69844=CARTESIAN_POINT('Ctrl Pts',(-20.8461018015119,-19.1187818254321,
-16.4770994536599));
#69845=CARTESIAN_POINT('Ctrl Pts',(-20.8349011937254,-19.2127900061834,
-16.4713270646499));
#69846=CARTESIAN_POINT('Ctrl Pts',(-20.833594094072,-19.2231123371005,-16.4706950869428));
#69847=CARTESIAN_POINT('Ctrl Pts',(-20.8312616504181,-19.240502273878,-16.4696334224317));
#69848=CARTESIAN_POINT('Ctrl Pts',(-20.8302765584432,-19.2475750071037,
-16.469202473263));
#69849=CARTESIAN_POINT('Ctrl Pts',(-20.8283990623356,-19.2605732870644,
-16.4684119901868));
#69850=CARTESIAN_POINT('Ctrl Pts',(-20.8275172529268,-19.2665002681227,
-16.4680521249301));
#69851=CARTESIAN_POINT('Ctrl Pts',(-20.8256463302589,-19.2787188236985,
-16.4673114273671));
#69852=CARTESIAN_POINT('Ctrl Pts',(-20.8246539659489,-19.2850098447147,
-16.4669307021733));
#69853=CARTESIAN_POINT('Ctrl Pts',(-20.8223696973859,-19.2990780288716,
-16.466080705912));
#69854=CARTESIAN_POINT('Ctrl Pts',(-20.8210627049252,-19.3068526727633,
-16.465611918897));
#69855=CARTESIAN_POINT('Ctrl Pts',(-20.8176411994243,-19.3265324415733,
-16.4644276122011));
#69856=CARTESIAN_POINT('Ctrl Pts',(-20.8154680485809,-19.3384271853317,
-16.4637139590921));
#69857=CARTESIAN_POINT('Ctrl Pts',(-20.8024833847127,-19.4062088330175,
-16.4596586629898));
#69858=CARTESIAN_POINT('Ctrl Pts',(-20.7895226652581,-19.4616632041659,
-16.4563862199873));
#69859=CARTESIAN_POINT('Ctrl Pts',(-20.7635221215107,-19.5556348933712,
-16.4508784060091));
#69860=CARTESIAN_POINT('Ctrl Pts',(-20.7515805991621,-19.5944203261352,
-16.4486161568553));
#69861=CARTESIAN_POINT('Ctrl Pts',(-20.7333849108257,-19.6479921359283,
-16.4454902009214));
#69862=CARTESIAN_POINT('Ctrl Pts',(-20.7280675950838,-19.6630832216733,
-16.4446094526583));
#69863=CARTESIAN_POINT('Ctrl Pts',(-20.7225805882177,-19.6781103526075,
-16.4437314133151));
#69864=CARTESIAN_POINT('Origin',(-18.734,-18.952,0.));
#69865=CARTESIAN_POINT('',(-20.7225805821192,-19.6781103693094,-15.6464962362309));
#69866=CARTESIAN_POINT('',(-20.7225805818996,-19.6781103699107,-15.8662165012922));
#69867=CARTESIAN_POINT('',(-20.7225805821191,-19.6781103693095,0.));
#69868=CARTESIAN_POINT('Ctrl Pts',(-20.7225805818996,-19.6781103699108,
-15.8662165012922));
#69869=CARTESIAN_POINT('Ctrl Pts',(-20.7307297073631,-19.6557925607626,
-15.8675067386898));
#69870=CARTESIAN_POINT('Ctrl Pts',(-20.7385063359538,-19.6333287725036,
-15.8687972801593));
#69871=CARTESIAN_POINT('Ctrl Pts',(-20.7729860297178,-19.5280199103041,
-15.8748265072091));
#69872=CARTESIAN_POINT('Ctrl Pts',(-20.7949379644017,-19.4437268313758,
-15.8795908542221));
#69873=CARTESIAN_POINT('Ctrl Pts',(-20.8189001336634,-19.3212038664771,
-15.8867187228425));
#69874=CARTESIAN_POINT('Ctrl Pts',(-20.8251640472988,-19.2838924378082,
-15.8889161159917));
#69875=CARTESIAN_POINT('Ctrl Pts',(-20.8314778232722,-19.2389374792607,
-15.891617064197));
#69876=CARTESIAN_POINT('Ctrl Pts',(-20.8324907022321,-19.2314335428028,
-15.8920696870342));
#69877=CARTESIAN_POINT('Ctrl Pts',(-20.8340004993622,-19.2197767627973,
-15.8927757821714));
#69878=CARTESIAN_POINT('Ctrl Pts',(-20.8345254155855,-19.2156275209463,
-15.8930277028585));
#69879=CARTESIAN_POINT('Ctrl Pts',(-20.8354748338075,-19.2079398824014,
-15.8934955857831));
#69880=CARTESIAN_POINT('Ctrl Pts',(-20.8359026977986,-19.204401959056,-15.8937113561156));
#69881=CARTESIAN_POINT('Ctrl Pts',(-20.836848273341,-19.1964140132555,-15.8941995263774));
#69882=CARTESIAN_POINT('Ctrl Pts',(-20.8373607906041,-19.1919634435997,
-15.8944722133263));
#69883=CARTESIAN_POINT('Ctrl Pts',(-20.8388276183908,-19.1788600437951,
-15.8952770454309));
#69884=CARTESIAN_POINT('Ctrl Pts',(-20.839742674446,-19.1702030376726,-15.8958113186995));
#69885=CARTESIAN_POINT('Ctrl Pts',(-20.8458591842089,-19.1087111214722,
-15.8996232153201));
#69886=CARTESIAN_POINT('Ctrl Pts',(-20.8491244442865,-19.0557070469998,
-15.9029969900621));
#69887=CARTESIAN_POINT('Ctrl Pts',(-20.8507874982691,-18.9862051756932,
-15.9074893528494));
#69888=CARTESIAN_POINT('Ctrl Pts',(-20.8509892979632,-18.9697651435171,
-15.9085570237302));
#69889=CARTESIAN_POINT('Ctrl Pts',(-20.8510113340041,-18.9345499588899,
-15.9108527723505));
#69890=CARTESIAN_POINT('Ctrl Pts',(-20.8507733234041,-18.9157761482131,
-15.9120820035659));
#69891=CARTESIAN_POINT('Ctrl Pts',(-20.8462294455872,-18.7409108018803,
-15.9235687182214));
#69892=CARTESIAN_POINT('Ctrl Pts',(-20.824913746761,-18.5857188053272,-15.9339903193705));
#69893=CARTESIAN_POINT('Ctrl Pts',(-20.785542695512,-18.4296163464068,-15.9442510920221));
#69894=CARTESIAN_POINT('Ctrl Pts',(-20.7843510914448,-18.4249587156732,
-15.9445570831285));
#69895=CARTESIAN_POINT('Ctrl Pts',(-20.7672392267998,-18.3590098563247,
-15.9488873945985));
#69896=CARTESIAN_POINT('Ctrl Pts',(-20.7485914678273,-18.2984545857325,
-15.9528337086067));
#69897=CARTESIAN_POINT('Ctrl Pts',(-20.723039946784,-18.2270409458947,-15.9574538815467));
#69898=CARTESIAN_POINT('Ctrl Pts',(-20.7187205985596,-18.2152980954052,
-15.9582125358089));
#69899=CARTESIAN_POINT('Ctrl Pts',(-20.711464542166,-18.1960984236054,-15.9594513604962));
#69900=CARTESIAN_POINT('Ctrl Pts',(-20.7085891943353,-18.1886188860803,
-15.9599335680101));
#69901=CARTESIAN_POINT('Ctrl Pts',(-20.7033484027647,-18.1752139482393,
-15.9607971315853));
#69902=CARTESIAN_POINT('Ctrl Pts',(-20.7009985212042,-18.1692826048676,
-15.9611790045827));
#69903=CARTESIAN_POINT('Ctrl Pts',(-20.695942226651,-18.1566865775832,-15.9619895093439));
#69904=CARTESIAN_POINT('Ctrl Pts',(-20.6932285809807,-18.1500248694498,
-15.962417891435));
#69905=CARTESIAN_POINT('Ctrl Pts',(-20.6858430804973,-18.1321554884538,
-15.9635663282357));
#69906=CARTESIAN_POINT('Ctrl Pts',(-20.6811086239729,-18.1209738573857,
-15.9642842555008));
#69907=CARTESIAN_POINT('Ctrl Pts',(-20.6571507113779,-18.0657200273455,
-15.9678291910116));
#69908=CARTESIAN_POINT('Ctrl Pts',(-20.6365250241544,-18.0222689096136,
-15.9706079109111));
#69909=CARTESIAN_POINT('Ctrl Pts',(-20.5374247689133,-17.8306367182849,
-15.982882583839));
#69910=CARTESIAN_POINT('Ctrl Pts',(-20.4430001204703,-17.6913983093555,
-15.9918006202372));
#69911=CARTESIAN_POINT('Ctrl Pts',(-20.2684487327962,-17.490185758686,-16.0063842130121));
#69912=CARTESIAN_POINT('Ctrl Pts',(-20.1986330781035,-17.4202432918067,
-16.0118768798071));
#69913=CARTESIAN_POINT('Ctrl Pts',(-20.116893153225,-17.3490684601606,-16.0182980400643));
#69914=CARTESIAN_POINT('Ctrl Pts',(-20.1095379792872,-17.3427522707442,
-16.0188757783208));
#69915=CARTESIAN_POINT('Ctrl Pts',(-20.0986146014658,-17.3335015200414,
-16.0197341610803));
#69916=CARTESIAN_POINT('Ctrl Pts',(-20.0950796391646,-17.330527658242,-16.0200120022496));
#69917=CARTESIAN_POINT('Ctrl Pts',(-20.0887912534383,-17.3252724735151,
-16.0205064146653));
#69918=CARTESIAN_POINT('Ctrl Pts',(-20.0860417539721,-17.3229865313253,
-16.0207226439304));
#69919=CARTESIAN_POINT('Ctrl Pts',(-20.0801385597367,-17.3181038385677,
-16.0211870247424));
#69920=CARTESIAN_POINT('Ctrl Pts',(-20.0769831838498,-17.315509286431,-16.0214353225418));
#69921=CARTESIAN_POINT('Ctrl Pts',(-20.0683014467751,-17.308412625049,-16.022118654952));
#69922=CARTESIAN_POINT('Ctrl Pts',(-20.0627598849563,-17.3039293174251,
-16.0225550070918));
#69923=CARTESIAN_POINT('Ctrl Pts',(-20.0330578005015,-17.2801465270536,
-16.0248942708288));
#69924=CARTESIAN_POINT('Ctrl Pts',(-20.0085005815772,-17.2613512374302,
-16.0268299549707));
#69925=CARTESIAN_POINT('Ctrl Pts',(-19.9329337739125,-17.2060969789132,
-16.0327693242548));
#69926=CARTESIAN_POINT('Ctrl Pts',(-19.8807099396329,-17.1713611346017,
-16.0368504395713));
#69927=CARTESIAN_POINT('Ctrl Pts',(-19.7118261973956,-17.069544292936,-16.0498094577686));
#69928=CARTESIAN_POINT('Ctrl Pts',(-19.5902576567293,-17.011223973896,-16.0587751100883));
#69929=CARTESIAN_POINT('Ctrl Pts',(-19.4256424332872,-16.9507535730585,
-16.0700685598907));
#69930=CARTESIAN_POINT('Ctrl Pts',(-19.3869105182043,-16.9377843483163,
-16.0726705063229));
#69931=CARTESIAN_POINT('Ctrl Pts',(-19.3014162312955,-16.9118825127892,
-16.078289482811));
#69932=CARTESIAN_POINT('Ctrl Pts',(-19.2545346260604,-16.8994199531673,
-16.0812910948842));
#69933=CARTESIAN_POINT('Ctrl Pts',(-19.1949880224102,-16.885762441544,-16.0850069640793));
#69934=CARTESIAN_POINT('Ctrl Pts',(-19.1826878327295,-16.8830565874611,
-16.0857694323499));
#69935=CARTESIAN_POINT('Ctrl Pts',(-19.1631556963317,-16.8789421971943,
-16.0869723028478));
#69936=CARTESIAN_POINT('Ctrl Pts',(-19.1559394293538,-16.8774614041765,
-16.0874150104652));
#69937=CARTESIAN_POINT('Ctrl Pts',(-19.1424773022615,-16.8747720968182,
-16.0882377754221));
#69938=CARTESIAN_POINT('Ctrl Pts',(-19.1362334589182,-16.8735540146271,
-16.0886181344525));
#69939=CARTESIAN_POINT('Ctrl Pts',(-19.1223512337462,-16.8709106955121,
-16.0894610799128));
#69940=CARTESIAN_POINT('Ctrl Pts',(-19.1147102805593,-16.8694993256313,
-16.0899232197061));
#69941=CARTESIAN_POINT('Ctrl Pts',(-19.0924792282726,-16.8655194452934,
-16.0912625979884));
#69942=CARTESIAN_POINT('Ctrl Pts',(-19.07786953696,-16.8630619395223,-16.0921363050671));
#69943=CARTESIAN_POINT('Ctrl Pts',(-18.9612384673987,-16.8447001116722,
-16.0990619156478));
#69944=CARTESIAN_POINT('Ctrl Pts',(-18.8581971845694,-16.8361244791702,
-16.1048707927129));
#69945=CARTESIAN_POINT('Ctrl Pts',(-18.5952941200334,-16.8335251301355,
-16.1193460039176));
#69946=CARTESIAN_POINT('Ctrl Pts',(-18.4360075589186,-16.8500086332339,
-16.1277742615311));
#69947=CARTESIAN_POINT('Ctrl Pts',(-18.2326901373384,-16.8946391933719,
-16.1395293310831));
#69948=CARTESIAN_POINT('Ctrl Pts',(-18.1856554523271,-16.9066730003033,
-16.1423242163451));
#69949=CARTESIAN_POINT('Ctrl Pts',(-18.1316341104387,-16.9224915547226,
-16.1456660586379));
#69950=CARTESIAN_POINT('Ctrl Pts',(-18.1242004327744,-16.9247127292859,
-16.1461288521409));
#69951=CARTESIAN_POINT('Ctrl Pts',(-18.1123335104085,-16.9283297263186,
-16.1468725918947));
#69952=CARTESIAN_POINT('Ctrl Pts',(-18.1078922821448,-16.9296993978238,
-16.1471520510458));
#69953=CARTESIAN_POINT('Ctrl Pts',(-18.1000301754268,-16.9321524469193,
-16.1476487975376));
#69954=CARTESIAN_POINT('Ctrl Pts',(-18.0966074987592,-16.933229910229,-16.147865736357));
#69955=CARTESIAN_POINT('Ctrl Pts',(-18.0893539728442,-16.9355336159061,
-16.148326962341));
#69956=CARTESIAN_POINT('Ctrl Pts',(-18.0855239340054,-16.9367620563027,
-16.1485713717932));
#69957=CARTESIAN_POINT('Ctrl Pts',(-18.0751862449485,-16.9401102715605,
-16.1492333693634));
#69958=CARTESIAN_POINT('Ctrl Pts',(-18.0686854010582,-16.942250681124,-16.1496521438467));
#69959=CARTESIAN_POINT('Ctrl Pts',(-18.0363464092235,-16.9530724261805,
-16.1517473348381));
#69960=CARTESIAN_POINT('Ctrl Pts',(-18.0106685216641,-16.9622202666219,
-16.1534490867683));
#69961=CARTESIAN_POINT('Ctrl Pts',(-17.9367563134362,-16.9901714554309,
-16.1584442879741));
#69962=CARTESIAN_POINT('Ctrl Pts',(-17.8890277863969,-17.010250796015,-16.1617909400697));
#69963=CARTESIAN_POINT('Ctrl Pts',(-17.7166886170026,-17.0903113315996,
-16.1742124396346));
#69964=CARTESIAN_POINT('Ctrl Pts',(-17.597288628506,-17.1607159740872,-16.1834585095198));
#69965=CARTESIAN_POINT('Ctrl Pts',(-17.4531469320556,-17.2659632502434,
-16.1950149431767));
#69966=CARTESIAN_POINT('Ctrl Pts',(-17.4213661164519,-17.29058581986,-16.1975929186163));
#69967=CARTESIAN_POINT('Ctrl Pts',(-17.344704883126,-17.3535538163037,-16.2038798760515));
#69968=CARTESIAN_POINT('Ctrl Pts',(-17.3006884029328,-17.3929008792986,
-16.2075501422267));
#69969=CARTESIAN_POINT('Ctrl Pts',(-17.2496029708767,-17.4425617087246,
-16.2118882697548));
#69970=CARTESIAN_POINT('Ctrl Pts',(-17.2409097805524,-17.4511602011974,
-16.212629434554));
#69971=CARTESIAN_POINT('Ctrl Pts',(-17.2267051619272,-17.4654556568296,
-16.213845546833));
#69972=CARTESIAN_POINT('Ctrl Pts',(-17.2211504544276,-17.4711090289222,
-16.2143224067282));
#69973=CARTESIAN_POINT('Ctrl Pts',(-17.2111873122963,-17.4813637021452,
-16.2151801361274));
#69974=CARTESIAN_POINT('Ctrl Pts',(-17.2067676778156,-17.485953944158,-16.2155614938385));
#69975=CARTESIAN_POINT('Ctrl Pts',(-17.1973631353017,-17.4958102032354,
-16.2163748935207));
#69976=CARTESIAN_POINT('Ctrl Pts',(-17.192384411972,-17.5010820288839,-16.2168066650069));
#69977=CARTESIAN_POINT('Ctrl Pts',(-17.1789621322447,-17.515441575901,-16.2179739357592));
#69978=CARTESIAN_POINT('Ctrl Pts',(-17.1705711219523,-17.5245781880762,
-16.2187071834209));
#69979=CARTESIAN_POINT('Ctrl Pts',(-17.1278099758911,-17.5719684084614,
-16.2224630341443));
#69980=CARTESIAN_POINT('Ctrl Pts',(-17.0947600209543,-17.6113932318482,
-16.2254299769808));
#69981=CARTESIAN_POINT('Ctrl Pts',(-16.9576006213985,-17.787675166661,-16.2381062496942));
#69982=CARTESIAN_POINT('Ctrl Pts',(-16.8689509324528,-17.9357130626752,
-16.2472181060822));
#69983=CARTESIAN_POINT('Ctrl Pts',(-16.7623787979088,-18.1757136384445,
-16.2616422174618));
#69984=CARTESIAN_POINT('Ctrl Pts',(-16.7309467633218,-18.2608529208552,
-16.2667142656139));
#69985=CARTESIAN_POINT('Ctrl Pts',(-16.7023147312639,-18.3569896908033,
-16.2726574334312));
#69986=CARTESIAN_POINT('Ctrl Pts',(-16.6996211110768,-18.3662655656631,
-16.2732330582019));
#69987=CARTESIAN_POINT('Ctrl Pts',(-16.6957351603995,-18.3799976229443,
-16.2740888894661));
#69988=CARTESIAN_POINT('Ctrl Pts',(-16.6944937228095,-18.384439941428,-16.2743663166008));
#69989=CARTESIAN_POINT('Ctrl Pts',(-16.6923158902063,-18.3923324411364,
-16.274860272318));
#69990=CARTESIAN_POINT('Ctrl Pts',(-16.6913737063379,-18.3957809740255,
-16.2750764612642));
#69991=CARTESIAN_POINT('Ctrl Pts',(-16.6893724302406,-18.4031796055299,
-16.2755410727289));
#69992=CARTESIAN_POINT('Ctrl Pts',(-16.6883160633632,-18.4071303319706,
-16.2757896431559));
#69993=CARTESIAN_POINT('Ctrl Pts',(-16.6854447442728,-18.417994888008,-16.2764744769912));
#69994=CARTESIAN_POINT('Ctrl Pts',(-16.6836533712204,-18.4249148134376,
-16.2769120673802));
#69995=CARTESIAN_POINT('Ctrl Pts',(-16.6742310377856,-18.4620874721685,
-16.2792697415396));
#69996=CARTESIAN_POINT('Ctrl Pts',(-16.6672349675675,-18.4924953491425,
-16.2812231993285));
#69997=CARTESIAN_POINT('Ctrl Pts',(-16.627713372978,-18.6834981951835,-16.2936015929701));
#69998=CARTESIAN_POINT('Ctrl Pts',(-16.6132535348419,-18.847258617052,-16.3046384230338));
#69999=CARTESIAN_POINT('Ctrl Pts',(-16.6210914435983,-19.1281630343,-16.3229964133678));
#70000=CARTESIAN_POINT('Ctrl Pts',(-16.6340762233565,-19.2448207436232,
-16.3304606218551));
#70001=CARTESIAN_POINT('Ctrl Pts',(-16.6594065554811,-19.3738475502771,
-16.3384894234507));
#70002=CARTESIAN_POINT('Ctrl Pts',(-16.6623021869892,-19.387845733046,-16.3393576801774));
#70003=CARTESIAN_POINT('Ctrl Pts',(-16.6671360999906,-19.4100765437877,
-16.3407323477502));
#70004=CARTESIAN_POINT('Ctrl Pts',(-16.6689822792973,-19.4183285510831,
-16.3412416890449));
#70005=CARTESIAN_POINT('Ctrl Pts',(-16.6723253280806,-19.4328619751784,
-16.3421371610188));
#70006=CARTESIAN_POINT('Ctrl Pts',(-16.6738015773789,-19.43914797841,-16.3425239482581));
#70007=CARTESIAN_POINT('Ctrl Pts',(-16.6769142396259,-19.4521347321018,
-16.3433219990456));
#70008=CARTESIAN_POINT('Ctrl Pts',(-16.6785546895061,-19.4588344434708,
-16.3437331274398));
#70009=CARTESIAN_POINT('Ctrl Pts',(-16.6828491576146,-19.4760095379292,
-16.3447856618007));
#70010=CARTESIAN_POINT('Ctrl Pts',(-16.6855507126369,-19.4864729157916,
-16.345425527474));
#70011=CARTESIAN_POINT('Ctrl Pts',(-16.6971569570993,-19.5300439431081,
-16.3480848022351));
#70012=CARTESIAN_POINT('Ctrl Pts',(-16.706785395659,-19.5629546020533,-16.350080713964));
#70013=CARTESIAN_POINT('Ctrl Pts',(-16.7339482874076,-19.6480700559076,
-16.3552209509689));
#70014=CARTESIAN_POINT('Ctrl Pts',(-16.7527277832449,-19.6998512037049,
-16.3583259643344));
#70015=CARTESIAN_POINT('Ctrl Pts',(-16.8147527759494,-19.8520706556725,
-16.3674659334321));
#70016=CARTESIAN_POINT('Ctrl Pts',(-16.863778822177,-19.949953268635,-16.3733521450796));
#70017=CARTESIAN_POINT('Ctrl Pts',(-16.9416095219262,-20.0792791547855,
-16.3815697480987));
#70018=CARTESIAN_POINT('Ctrl Pts',(-16.9641216557007,-20.1143047773691,
-16.3838450139904));
#70019=CARTESIAN_POINT('Ctrl Pts',(-17.0311327162433,-20.2120989320846,
-16.3904026078436));
#70020=CARTESIAN_POINT('Ctrl Pts',(-17.0780359042314,-20.2731307736757,
-16.3947452003717));
#70021=CARTESIAN_POINT('Ctrl Pts',(-17.1343438796865,-20.3386793683199,
-16.3998664796256));
#70022=CARTESIAN_POINT('Ctrl Pts',(-17.1405868348899,-20.3458485754957,
-16.4004331242079));
#70023=CARTESIAN_POINT('Ctrl Pts',(-17.1499104684294,-20.3564110357957,
-16.4012781059771));
#70024=CARTESIAN_POINT('Ctrl Pts',(-17.1529543207881,-20.3598368374339,
-16.4015537645834));
#70025=CARTESIAN_POINT('Ctrl Pts',(-17.1583904642936,-20.3659152557592,
-16.4020457781542));
#70026=CARTESIAN_POINT('Ctrl Pts',(-17.1607783691927,-20.3685717276609,
-16.402261803503));
#70027=CARTESIAN_POINT('Ctrl Pts',(-17.1659275891408,-20.3742709999359,
-16.4027274394942));
#70028=CARTESIAN_POINT('Ctrl Pts',(-17.1686910023114,-20.3773117638076,
-16.4029772052739));
#70029=CARTESIAN_POINT('Ctrl Pts',(-17.1763453185439,-20.3856851997488,
-16.40366863207));
#70030=CARTESIAN_POINT('Ctrl Pts',(-17.1812546833882,-20.3910008119867,
-16.4041116619195));
#70031=CARTESIAN_POINT('Ctrl Pts',(-17.2083326956934,-20.4200196081166,
-16.406552299704));
#70032=CARTESIAN_POINT('Ctrl Pts',(-17.2310156302216,-20.4432343914375,
-16.4085860627614));
#70033=CARTESIAN_POINT('Ctrl Pts',(-17.3706243523507,-20.5796949415688,
-16.4209903017239));
#70034=CARTESIAN_POINT('Ctrl Pts',(-17.4997570231484,-20.6796655268624,
-16.431952013662));
#70035=CARTESIAN_POINT('Ctrl Pts',(-17.7390557556664,-20.8242776971859,
-16.4502154948345));
#70036=CARTESIAN_POINT('Ctrl Pts',(-17.8438866526415,-20.8763294579752,
-16.4576574610546));
#70037=CARTESIAN_POINT('Ctrl Pts',(-17.9657765122672,-20.924745785803,-16.4656657234253));
#70038=CARTESIAN_POINT('Ctrl Pts',(-17.9791123996447,-20.9298872538807,
-16.4665338655643));
#70039=CARTESIAN_POINT('Ctrl Pts',(-18.0004192664867,-20.9378549290987,
-16.4679083865762));
#70040=CARTESIAN_POINT('Ctrl Pts',(-18.0083566990605,-20.9407690401476,
-16.4684176949259));
#70041=CARTESIAN_POINT('Ctrl Pts',(-18.0223859534902,-20.9458245007206,
-16.4693131285768));
#70042=CARTESIAN_POINT('Ctrl Pts',(-18.0284704724675,-20.9479856657993,
-16.4696999102613));
#70043=CARTESIAN_POINT('Ctrl Pts',(-18.0410752305636,-20.9523979210925,
-16.4704979683508));
#70044=CARTESIAN_POINT('Ctrl Pts',(-18.0475967820586,-20.9546450516606,
-16.4709091095094));
#70045=CARTESIAN_POINT('Ctrl Pts',(-18.0643639933708,-20.9603310021628,
-16.4719617153794));
#70046=CARTESIAN_POINT('Ctrl Pts',(-18.0746252935829,-20.9637233405008,
-16.4726016393864));
#70047=CARTESIAN_POINT('Ctrl Pts',(-18.1175531244837,-20.9775513388981,
-16.475261480885));
#70048=CARTESIAN_POINT('Ctrl Pts',(-18.1504458883981,-20.9872714246678,
-16.4772578882314));
#70049=CARTESIAN_POINT('Ctrl Pts',(-18.2367445345147,-21.0105090455725,
-16.482399690011));
#70050=CARTESIAN_POINT('Ctrl Pts',(-18.2904683501457,-21.0227493350961,
-16.4855057411379));
#70051=CARTESIAN_POINT('Ctrl Pts',(-18.4520695669314,-21.0529892443179,
-16.4946475209051));
#70052=CARTESIAN_POINT('Ctrl Pts',(-18.5609267548231,-21.064743976899,-16.5005345114323));
#70053=CARTESIAN_POINT('Ctrl Pts',(-18.7135619749919,-21.0693457143934,
-16.5088482751542));
#70054=CARTESIAN_POINT('Ctrl Pts',(-18.7569483798989,-21.0693199480965,
-16.5112195249736));
#70055=CARTESIAN_POINT('Ctrl Pts',(-18.8292945691319,-21.0670530332496,
-16.5152274137375));
#70056=CARTESIAN_POINT('Ctrl Pts',(-18.8582643923496,-21.0655488262737,
-16.5168468049708));
#70057=CARTESIAN_POINT('Ctrl Pts',(-18.934671416717,-21.0600052256225,-16.5211766017069));
#70058=CARTESIAN_POINT('Ctrl Pts',(-18.9820161163156,-21.054960367503,-16.5239194265345));
#70059=CARTESIAN_POINT('Ctrl Pts',(-19.0367909684201,-21.0472484879392,
-16.5272036879119));
#70060=CARTESIAN_POINT('Ctrl Pts',(-19.0444293916131,-21.0461304127202,
-16.5276642081705));
#70061=CARTESIAN_POINT('Ctrl Pts',(-19.056645123054,-21.0442740308887,-16.5284049847111));
#70062=CARTESIAN_POINT('Ctrl Pts',(-19.0612264989245,-21.0435624095942,
-16.5286837725493));
#70063=CARTESIAN_POINT('Ctrl Pts',(-19.0693479602099,-21.0422735732448,
-16.5291797591694));
#70064=CARTESIAN_POINT('Ctrl Pts',(-19.0728889590211,-21.0417024043409,
-16.5293966131512));
#70065=CARTESIAN_POINT('Ctrl Pts',(-19.0804041624123,-21.0404705854899,
-16.5298581488512));
#70066=CARTESIAN_POINT('Ctrl Pts',(-19.0843778756344,-21.039807599812,-16.5301029553359));
#70067=CARTESIAN_POINT('Ctrl Pts',(-19.0951257728073,-21.0379828416812,
-16.5307671253537));
#70068=CARTESIAN_POINT('Ctrl Pts',(-19.1018961622764,-21.0367994268902,
-16.5311876883415));
#70069=CARTESIAN_POINT('Ctrl Pts',(-19.1358330208706,-21.0306970532555,
-16.5333063336567));
#70070=CARTESIAN_POINT('Ctrl Pts',(-19.1629058272887,-21.0252802121215,
-16.5350304228148));
#70071=CARTESIAN_POINT('Ctrl Pts',(-19.2413869743396,-21.0079745173343,
-16.5401125336286));
#70072=CARTESIAN_POINT('Ctrl Pts',(-19.2924644680803,-20.9946917149017,
-16.5435258094916));
#70073=CARTESIAN_POINT('Ctrl Pts',(-19.4895943261432,-20.9354813986299,
-16.5569879476815));
#70074=CARTESIAN_POINT('Ctrl Pts',(-19.6310094190138,-20.8756691335443,
-16.5672342660921));
#70075=CARTESIAN_POINT('Ctrl Pts',(-19.8353826395793,-20.7617476874904,
-16.5822648906721));
#70076=CARTESIAN_POINT('Ctrl Pts',(-19.903719246692,-20.7183493440658,-16.5873428662116));
#70077=CARTESIAN_POINT('Ctrl Pts',(-19.9802669652236,-20.6633405086758,
-16.5930915676057));
#70078=CARTESIAN_POINT('Ctrl Pts',(-19.9910481576296,-20.6554370042672,
-16.5939028141868));
#70079=CARTESIAN_POINT('Ctrl Pts',(-20.008308359053,-20.6425307409812,-16.5952043446949));
#70080=CARTESIAN_POINT('Ctrl Pts',(-20.0148343478352,-20.6375916932928,
-16.5956970935598));
#70081=CARTESIAN_POINT('Ctrl Pts',(-20.026272329459,-20.6288303313179,-16.5965619293752));
#70082=CARTESIAN_POINT('Ctrl Pts',(-20.0311963830989,-20.6250239921982,
-16.5969346386755));
#70083=CARTESIAN_POINT('Ctrl Pts',(-20.0414236845828,-20.6170458958003,
-16.5977096249164));
#70084=CARTESIAN_POINT('Ctrl Pts',(-20.0467239238317,-20.6128703825253,
-16.5981117469378));
#70085=CARTESIAN_POINT('Ctrl Pts',(-20.0603108395095,-20.6020609780745,
-16.5991438941817));
#70086=CARTESIAN_POINT('Ctrl Pts',(-20.068567811867,-20.5953899221138,-16.5997724252275));
#70087=CARTESIAN_POINT('Ctrl Pts',(-20.086430415661,-20.5807347760682,-16.6011351766353));
#70088=CARTESIAN_POINT('Ctrl Pts',(-20.0960163054245,-20.5727271804937,
-16.6018684283294));
#70089=CARTESIAN_POINT('Ctrl Pts',(-20.123608919686,-20.5492599225391,-16.603985285176));
#70090=CARTESIAN_POINT('Ctrl Pts',(-20.1414275846905,-20.5335814450706,
-16.605360082202));
#70091=CARTESIAN_POINT('Ctrl Pts',(-20.2021858590854,-20.4782806373543,
-16.610080719691));
#70092=CARTESIAN_POINT('Ctrl Pts',(-20.243747922432,-20.437181557718,-16.613367421976));
#70093=CARTESIAN_POINT('Ctrl Pts',(-20.3971128987807,-20.2724242825409,
-16.6258507220206));
#70094=CARTESIAN_POINT('Ctrl Pts',(-20.4958546396415,-20.13746453344,-16.6346274445503));
#70095=CARTESIAN_POINT('Ctrl Pts',(-20.6057404058206,-19.9427180856376,
-16.6471659685301));
#70096=CARTESIAN_POINT('Ctrl Pts',(-20.631719340746,-19.891997105722,-16.6504265390946));
#70097=CARTESIAN_POINT('Ctrl Pts',(-20.6593362816642,-19.832254327075,-16.6543312422468));
#70098=CARTESIAN_POINT('Ctrl Pts',(-20.6630028482097,-19.8241900499486,
-16.6548596342938));
#70099=CARTESIAN_POINT('Ctrl Pts',(-20.6684606891082,-19.8119832609207,
-16.6556617934192));
#70100=CARTESIAN_POINT('Ctrl Pts',(-20.6702895594041,-19.8078575278895,
-16.6559333136565));
#70101=CARTESIAN_POINT('Ctrl Pts',(-20.6735399307298,-19.8004612978634,
-16.6564208415383));
#70102=CARTESIAN_POINT('Ctrl Pts',(-20.6749663723949,-19.7971930299199,
-16.6566365430581));
#70103=CARTESIAN_POINT('Ctrl Pts',(-20.678038007097,-19.7901065040981,-16.6571048446689));
#70104=CARTESIAN_POINT('Ctrl Pts',(-20.6796801896291,-19.7862870514682,
-16.6573576178657));
#70105=CARTESIAN_POINT('Ctrl Pts',(-20.684236790219,-19.7756025047067,-16.6580657099068));
#70106=CARTESIAN_POINT('Ctrl Pts',(-20.687126163031,-19.7687268889667,-16.658522505925));
#70107=CARTESIAN_POINT('Ctrl Pts',(-20.70143825064,-19.734159229708,-16.6608242189666));
#70108=CARTESIAN_POINT('Ctrl Pts',(-20.712307776493,-19.7062442490166,-16.6626994153792));
#70109=CARTESIAN_POINT('Ctrl Pts',(-20.7225805820307,-19.6781103695518,
-16.6645990581914));
#70110=CARTESIAN_POINT('Ctrl Pts',(-20.7225805882177,-19.6781103526075,
-16.4437314133151));
#70111=CARTESIAN_POINT('Ctrl Pts',(-20.6965443416094,-19.7494151817003,
-16.4395650527784));
#70112=CARTESIAN_POINT('Ctrl Pts',(-20.6666873095021,-19.8192801308043,
-16.4354619668037));
#70113=CARTESIAN_POINT('Ctrl Pts',(-20.5942956802539,-19.9662562803097,
-16.4265492207356));
#70114=CARTESIAN_POINT('Ctrl Pts',(-20.5505851114218,-20.0426107945465,
-16.42173972251));
#70115=CARTESIAN_POINT('Ctrl Pts',(-20.4813387103453,-20.1478027480543,
-16.414551017801));
#70116=CARTESIAN_POINT('Ctrl Pts',(-20.4595656891349,-20.1790123990853,
-16.412341193437));
#70117=CARTESIAN_POINT('Ctrl Pts',(-20.4324595281259,-20.2157174357495,
-16.4096264675339));
#70118=CARTESIAN_POINT('Ctrl Pts',(-20.4279211758614,-20.2217943030754,
-16.4091731046042));
#70119=CARTESIAN_POINT('Ctrl Pts',(-20.4208281426725,-20.2311861990604,
-16.4084661017703));
#70120=CARTESIAN_POINT('Ctrl Pts',(-20.4182960678511,-20.2345183312157,
-16.4082140198899));
#70121=CARTESIAN_POINT('Ctrl Pts',(-20.413589689593,-20.2406738041639,-16.407745990402));
#70122=CARTESIAN_POINT('Ctrl Pts',(-20.4114181316746,-20.2434991714577,
-16.4075302356777));
#70123=CARTESIAN_POINT('Ctrl Pts',(-20.4065025452937,-20.2498614236785,
-16.4070422968037));
#70124=CARTESIAN_POINT('Ctrl Pts',(-20.403754442111,-20.2533950750197,-16.4067698268464));
#70125=CARTESIAN_POINT('Ctrl Pts',(-20.3956392669153,-20.2637619622676,
-16.4059662150643));
#70126=CARTESIAN_POINT('Ctrl Pts',(-20.390241384442,-20.2705708056536,-16.4054329545714));
#70127=CARTESIAN_POINT('Ctrl Pts',(-20.3519510790968,-20.318263787291,-16.4016602557134));
#70128=CARTESIAN_POINT('Ctrl Pts',(-20.3175931800649,-20.357942416745,-16.3983268976479));
#70129=CARTESIAN_POINT('Ctrl Pts',(-20.2680017203592,-20.4110876587015,
-16.3936317155812));
#70130=CARTESIAN_POINT('Ctrl Pts',(-20.2539921342721,-20.4256763379892,
-16.3923172380323));
#70131=CARTESIAN_POINT('Ctrl Pts',(-20.1944852553819,-20.4858916029021,
-16.3867903869416));
#70132=CARTESIAN_POINT('Ctrl Pts',(-20.1471268370527,-20.5296288550271,
-16.3825280283716));
#70133=CARTESIAN_POINT('Ctrl Pts',(-20.0268922266698,-20.6309061502357,
-16.372140645233));
#70134=CARTESIAN_POINT('Ctrl Pts',(-19.9520786154108,-20.6859501140268,
-16.3660355233576));
#70135=CARTESIAN_POINT('Ctrl Pts',(-19.8280107558721,-20.7652274675031,
-16.3565767560004));
#70136=CARTESIAN_POINT('Ctrl Pts',(-19.781014536084,-20.7927647155573,-16.3531305809863));
#70137=CARTESIAN_POINT('Ctrl Pts',(-19.7130843996956,-20.8291236711577,
-16.3483426168123));
#70138=CARTESIAN_POINT('Ctrl Pts',(-19.6929933449978,-20.8394669174303,
-16.3469494302334));
#70139=CARTESIAN_POINT('Ctrl Pts',(-19.6573339834099,-20.8571086029881,
-16.34451617133));
#70140=CARTESIAN_POINT('Ctrl Pts',(-19.6418354483742,-20.8645426165517,
-16.3434714780255));
#70141=CARTESIAN_POINT('Ctrl Pts',(-19.6187996745499,-20.8752488117673,
-16.3419372810226));
#70142=CARTESIAN_POINT('Ctrl Pts',(-19.6113314609758,-20.8786670616894,
-16.3414427414028));
#70143=CARTESIAN_POINT('Ctrl Pts',(-19.5982633387782,-20.8845566857527,
-16.3405822779501));
#70144=CARTESIAN_POINT('Ctrl Pts',(-19.5926722919433,-20.8870473789219,
-16.3402156928396));
#70145=CARTESIAN_POINT('Ctrl Pts',(-19.5815134480694,-20.8919605208084,
-16.3394871056638));
#70146=CARTESIAN_POINT('Ctrl Pts',(-19.5759458758095,-20.894383332492,-16.3391250938649));
#70147=CARTESIAN_POINT('Ctrl Pts',(-19.5626185698565,-20.9001148386649,
-16.3382620884902));
#70148=CARTESIAN_POINT('Ctrl Pts',(-19.554849294018,-20.9034011885252,-16.3377618588597));
#70149=CARTESIAN_POINT('Ctrl Pts',(-19.52678593254,-20.9150745393023,-16.3359651047281));
#70150=CARTESIAN_POINT('Ctrl Pts',(-19.5063808511285,-20.923192292935,-16.3346776783996));
#70151=CARTESIAN_POINT('Ctrl Pts',(-19.3109591509058,-20.9974363318907,
-16.3225174746201));
#70152=CARTESIAN_POINT('Ctrl Pts',(-19.1280358034047,-21.0404044882605,
-16.3125178271639));
#70153=CARTESIAN_POINT('Ctrl Pts',(-18.8630650279926,-21.0665439589387,
-16.2979982313434));
#70154=CARTESIAN_POINT('Ctrl Pts',(-18.7839281003975,-21.0698902634106,
-16.2936425055498));
#70155=CARTESIAN_POINT('Ctrl Pts',(-18.6690381780632,-21.0683052405551,
-16.2870682099507));
#70156=CARTESIAN_POINT('Ctrl Pts',(-18.6333003361813,-21.0669059425486,
-16.2849876505455));
#70157=CARTESIAN_POINT('Ctrl Pts',(-18.5901830977223,-21.0641224396186,
-16.2824162662473));
#70158=CARTESIAN_POINT('Ctrl Pts',(-18.5827513630383,-21.0636032646771,
-16.2819708562686));
#70159=CARTESIAN_POINT('Ctrl Pts',(-18.5711785764213,-21.0627333925416,
-16.2812736108339));
#70160=CARTESIAN_POINT('Ctrl Pts',(-18.5670354706511,-21.0624097032623,
-16.281023265122));
#70161=CARTESIAN_POINT('Ctrl Pts',(-18.559338781334,-21.0617855760697,-16.2805567962744));
#70162=CARTESIAN_POINT('Ctrl Pts',(-18.5557849942619,-21.0614883572606,
-16.2803408554299));
#70163=CARTESIAN_POINT('Ctrl Pts',(-18.5477332527692,-21.0607944631246,
-16.2798503427349));
#70164=CARTESIAN_POINT('Ctrl Pts',(-18.5432358284837,-21.0603923778133,
-16.2795754716863));
#70165=CARTESIAN_POINT('Ctrl Pts',(-18.5316183722626,-21.0593162615627,
-16.2788632089119));
#70166=CARTESIAN_POINT('Ctrl Pts',(-18.5245004749634,-21.0586205389605,
-16.2784246434546));
#70167=CARTESIAN_POINT('Ctrl Pts',(-18.4806283489905,-21.054107811997,-16.2757086713008));
#70168=CARTESIAN_POINT('Ctrl Pts',(-18.4439781266975,-21.0493653420743,
-16.2733843522618));
#70169=CARTESIAN_POINT('Ctrl Pts',(-18.2390314256798,-21.0173714603862,
-16.2601434386274));
#70170=CARTESIAN_POINT('Ctrl Pts',(-18.0743837399871,-20.9708270668219,
-16.2486402118437));
#70171=CARTESIAN_POINT('Ctrl Pts',(-17.8293240934374,-20.868325234724,-16.2313797227007));
#70172=CARTESIAN_POINT('Ctrl Pts',(-17.7441172019323,-20.8257334837867,
-16.225335611227));
#70173=CARTESIAN_POINT('Ctrl Pts',(-17.6436334443798,-20.7667303196802,
-16.2181781335989));
#70174=CARTESIAN_POINT('Ctrl Pts',(-17.6253762065773,-20.7556348565989,
-16.2168760293727));
#70175=CARTESIAN_POINT('Ctrl Pts',(-17.5996659066338,-20.739472028513,-16.2150394312111));
#70176=CARTESIAN_POINT('Ctrl Pts',(-17.5920728779454,-20.7346307918136,
-16.2144966541862));
#70177=CARTESIAN_POINT('Ctrl Pts',(-17.5790311576359,-20.7261980032417,
-16.213563661872));
#70178=CARTESIAN_POINT('Ctrl Pts',(-17.5735678025254,-20.7226294638018,
-16.2131725973743));
#70179=CARTESIAN_POINT('Ctrl Pts',(-17.5631414715522,-20.7157502363238,
-16.2124258240154));
#70180=CARTESIAN_POINT('Ctrl Pts',(-17.5581758275329,-20.7124437242739,
-16.2120699637226));
#70181=CARTESIAN_POINT('Ctrl Pts',(-17.5453058330529,-20.7037951341314,
-16.2111470739568));
#70182=CARTESIAN_POINT('Ctrl Pts',(-17.5374234418328,-20.698420499042,-16.2105812781564));
#70183=CARTESIAN_POINT('Ctrl Pts',(-17.5106998882713,-20.6799330878844,
-16.2086609029701));
#70184=CARTESIAN_POINT('Ctrl Pts',(-17.4920353678397,-20.6665669519341,
-16.2073159784082));
#70185=CARTESIAN_POINT('Ctrl Pts',(-17.3322184999601,-20.5481386973109,
-16.1957569848153));
#70186=CARTESIAN_POINT('Ctrl Pts',(-17.2044585721606,-20.4261641064983,
-16.1862985668844));
#70187=CARTESIAN_POINT('Ctrl Pts',(-17.0384864671159,-20.2226040308097,
-16.1720066095259));
#70188=CARTESIAN_POINT('Ctrl Pts',(-16.9878986156312,-20.152136793481,-16.1672607827379));
#70189=CARTESIAN_POINT('Ctrl Pts',(-16.9216892225718,-20.0468254857366,
-16.1601578865959));
#70190=CARTESIAN_POINT('Ctrl Pts',(-16.9024621345172,-20.0143473296375,
-16.1579656194571));
#70191=CARTESIAN_POINT('Ctrl Pts',(-16.8804352765808,-19.9747629606103,
-16.1552703528791));
#70192=CARTESIAN_POINT('Ctrl Pts',(-16.8767914847811,-19.9681312831427,
-16.1548180366995));
#70193=CARTESIAN_POINT('Ctrl Pts',(-16.8711895947806,-19.9578050888675,
-16.1541123176822));
#70194=CARTESIAN_POINT('Ctrl Pts',(-16.8692067153094,-19.9541239879695,
-16.1538604638047));
#70195=CARTESIAN_POINT('Ctrl Pts',(-16.8655539493425,-19.9472944574292,
-16.1533926415227));
#70196=CARTESIAN_POINT('Ctrl Pts',(-16.8638811029683,-19.9441476763009,
-16.1531768646174));
#70197=CARTESIAN_POINT('Ctrl Pts',(-16.8601226002057,-19.9370343010358,
-16.1526885979885));
#70198=CARTESIAN_POINT('Ctrl Pts',(-16.8580416005881,-19.9330653222381,
-16.1524158207411));
#70199=CARTESIAN_POINT('Ctrl Pts',(-16.8519522145636,-19.9213611474503,
-16.1516104805792));
#70200=CARTESIAN_POINT('Ctrl Pts',(-16.8479790138307,-19.9136078902488,
-16.1510757856137));
#70201=CARTESIAN_POINT('Ctrl Pts',(-16.8200772633822,-19.8583225891709,
-16.1472557105644));
#70202=CARTESIAN_POINT('Ctrl Pts',(-16.7979026066462,-19.8099316589153,
-16.1438737312689));
#70203=CARTESIAN_POINT('Ctrl Pts',(-16.7705880070477,-19.7438566544947,
-16.1392532703864));
#70204=CARTESIAN_POINT('Ctrl Pts',(-16.7638192297955,-19.726862130293,-16.138064623739));
#70205=CARTESIAN_POINT('Ctrl Pts',(-16.7400954038232,-19.664976871626,-16.1337399864725));
#70206=CARTESIAN_POINT('Ctrl Pts',(-16.7244478887265,-19.6196014091021,
-16.1305765881988));
#70207=CARTESIAN_POINT('Ctrl Pts',(-16.678233488877,-19.4691811711211,-16.1201818439999));
#70208=CARTESIAN_POINT('Ctrl Pts',(-16.6542595794201,-19.3622871688752,
-16.1129494699686));
#70209=CARTESIAN_POINT('Ctrl Pts',(-16.6307936785877,-19.1994824469219,
-16.1023767144949));
#70210=CARTESIAN_POINT('Ctrl Pts',(-16.6250650848887,-19.1446622344003,
-16.0988879529153));
#70211=CARTESIAN_POINT('Ctrl Pts',(-16.6192508866047,-19.055449097107,-16.0933309111094));
#70212=CARTESIAN_POINT('Ctrl Pts',(-16.6178522780413,-19.0211705386633,
-16.091224201238));
#70213=CARTESIAN_POINT('Ctrl Pts',(-16.6171091901768,-18.9760648108973,
-16.0884878423123));
#70214=CARTESIAN_POINT('Ctrl Pts',(-16.6170139158796,-18.965256781772,-16.087834855556));
#70215=CARTESIAN_POINT('Ctrl Pts',(-16.6169934382055,-18.9475503969162,
-16.0867693773816));
#70216=CARTESIAN_POINT('Ctrl Pts',(-16.6170191745592,-18.9406523959966,
-16.0863553566392));
#70217=CARTESIAN_POINT('Ctrl Pts',(-16.6171342735599,-18.9272980564383,
-16.0855558439122));
#70218=CARTESIAN_POINT('Ctrl Pts',(-16.6172194597147,-18.9208417669398,
-16.0851702256111));
#70219=CARTESIAN_POINT('Ctrl Pts',(-16.6174844047218,-18.9059324582976,
-16.0842817947634));
#70220=CARTESIAN_POINT('Ctrl Pts',(-16.6176852682019,-18.8974798881866,
-16.0837796483325));
#70221=CARTESIAN_POINT('Ctrl Pts',(-16.6183618392589,-18.8747446725737,
-16.0824329984989));
#70222=CARTESIAN_POINT('Ctrl Pts',(-16.6189315397412,-18.860465109764,-16.0815914367793));
#70223=CARTESIAN_POINT('Ctrl Pts',(-16.6254872555825,-18.7294624991767,
-16.0739072700658));
#70224=CARTESIAN_POINT('Ctrl Pts',(-16.6409851955418,-18.6134099410587,
-16.0673815790405));
#70225=CARTESIAN_POINT('Ctrl Pts',(-16.7008296409307,-18.3400803476614,
-16.0520640353285));
#70226=CARTESIAN_POINT('Ctrl Pts',(-16.7539192634356,-18.1855173050976,
-16.0434557340808));
#70227=CARTESIAN_POINT('Ctrl Pts',(-16.8381356195767,-18.0094334670877,
-16.0322460479717));
#70228=CARTESIAN_POINT('Ctrl Pts',(-16.8527443984693,-17.980603828165,-16.0303608616284));
#70229=CARTESIAN_POINT('Ctrl Pts',(-16.8714195007549,-17.9457519657349,
-16.0280065440628));
#70230=CARTESIAN_POINT('Ctrl Pts',(-16.8748651898488,-17.9393998929047,
-16.0275743307229));
#70231=CARTESIAN_POINT('Ctrl Pts',(-16.8803199322535,-17.9294658575846,
-16.0268932914705));
#70232=CARTESIAN_POINT('Ctrl Pts',(-16.8823070391383,-17.9258718189221,
-16.0266458449649));
#70233=CARTESIAN_POINT('Ctrl Pts',(-16.8860421809167,-17.9191623260885,
-16.0261818868966));
#70234=CARTESIAN_POINT('Ctrl Pts',(-16.8877876479322,-17.9160455067061,
-16.025965539632));
#70235=CARTESIAN_POINT('Ctrl Pts',(-16.8917918282189,-17.9089376423198,
-16.0254702946773));
#70236=CARTESIAN_POINT('Ctrl Pts',(-16.8940556183048,-17.9049495229261,
-16.0251910736221));
#70237=CARTESIAN_POINT('Ctrl Pts',(-16.8999983905922,-17.8945589266312,
-16.0244601380707));
#70238=CARTESIAN_POINT('Ctrl Pts',(-16.9036979083874,-17.8881683513176,
-16.0240071475843));
#70239=CARTESIAN_POINT('Ctrl Pts',(-16.9281580618464,-17.8464209629312,
-16.0210259776634));
#70240=CARTESIAN_POINT('Ctrl Pts',(-16.9499072548813,-17.8116567705678,
-16.0184400296505));
#70241=CARTESIAN_POINT('Ctrl Pts',(-16.9784220097713,-17.7688925822809,
-16.0151478810514));
#70242=CARTESIAN_POINT('Ctrl Pts',(-16.9842574587583,-17.7602792799255,
-16.0144789710384));
#70243=CARTESIAN_POINT('Ctrl Pts',(-16.9905359304933,-17.7511575926876,
-16.0137646197196));
#70244=CARTESIAN_POINT('Ctrl Pts',(-16.9909160501452,-17.7506058962115,
-16.0137213910916));
#70245=CARTESIAN_POINT('Ctrl Pts',(-17.0042631372199,-17.7312539256193,
-16.0122042346666));
#70246=CARTESIAN_POINT('Ctrl Pts',(-17.0175329087981,-17.712664990839,-16.010719851013));
#70247=CARTESIAN_POINT('Ctrl Pts',(-17.0582332092904,-17.6575578589333,
-16.0062449637163));
#70248=CARTESIAN_POINT('Ctrl Pts',(-17.0865470416795,-17.6217092975655,
-16.0032337948508));
#70249=CARTESIAN_POINT('Ctrl Pts',(-17.1865154718374,-17.503228617464,-15.9929935042399));
#70250=CARTESIAN_POINT('Ctrl Pts',(-17.2634088020367,-17.425234831801,-15.9857629243905));
#70251=CARTESIAN_POINT('Ctrl Pts',(-17.3875660012394,-17.3174246452061,
-15.9751939373817));
#70252=CARTESIAN_POINT('Ctrl Pts',(-17.4305385756909,-17.2829552916756,
-15.9717071375522));
#70253=CARTESIAN_POINT('Ctrl Pts',(-17.5023719887934,-17.2298045860117,
-15.9661528545762));
#70254=CARTESIAN_POINT('Ctrl Pts',(-17.5304270146847,-17.2100824109653,
-15.9640469893386));
#70255=CARTESIAN_POINT('Ctrl Pts',(-17.5679391598864,-17.1850512459489,
-15.9613115503641));
#70256=CARTESIAN_POINT('Ctrl Pts',(-17.5769741543946,-17.1791218367659,
-15.9606586585461));
#70257=CARTESIAN_POINT('Ctrl Pts',(-17.5918497696444,-17.1695215490091,
-15.9595932955746));
#70258=CARTESIAN_POINT('Ctrl Pts',(-17.5976635479298,-17.1658096276162,
-15.9591792957351));
#70259=CARTESIAN_POINT('Ctrl Pts',(-17.6089545764444,-17.1586780862025,
-15.9583797959415));
#70260=CARTESIAN_POINT('Ctrl Pts',(-17.6144295271651,-17.155254984882,-15.9579941698146));
#70261=CARTESIAN_POINT('Ctrl Pts',(-17.6271101524313,-17.1474071475838,
-15.9571056817313));
#70262=CARTESIAN_POINT('Ctrl Pts',(-17.6343268775291,-17.143000407816,-15.9566034861661));
#70263=CARTESIAN_POINT('Ctrl Pts',(-17.6538130472162,-17.131261292063,-15.955256617545));
#70264=CARTESIAN_POINT('Ctrl Pts',(-17.6661308009899,-17.1240096596888,
-15.9544148876857));
#70265=CARTESIAN_POINT('Ctrl Pts',(-17.780028306882,-17.0585008084712,-15.9467174988472));
#70266=CARTESIAN_POINT('Ctrl Pts',(-17.8862102738099,-17.0086371804574,
-15.9401800616163));
#70267=CARTESIAN_POINT('Ctrl Pts',(-18.1493513031603,-16.9107625393754,
-15.9248116845903));
#70268=CARTESIAN_POINT('Ctrl Pts',(-18.3087952433243,-16.8716987866076,
-15.9161664348669));
#70269=CARTESIAN_POINT('Ctrl Pts',(-18.5023526822931,-16.8474765297415,
-15.9049530743373));
#70270=CARTESIAN_POINT('Ctrl Pts',(-18.5336629784919,-16.8442655869463,
-15.9031159586999));
#70271=CARTESIAN_POINT('Ctrl Pts',(-18.5721758991528,-16.8411818331747,
-15.900815151354));
#70272=CARTESIAN_POINT('Ctrl Pts',(-18.5793232726317,-16.8406460553281,
-15.9003864256964));
#70273=CARTESIAN_POINT('Ctrl Pts',(-18.5905569835468,-16.8398613065372,
-15.8997096723339));
#70274=CARTESIAN_POINT('Ctrl Pts',(-18.5946416339385,-16.8395878705736,
-15.8994629954906));
#70275=CARTESIAN_POINT('Ctrl Pts',(-18.6022940441297,-16.8390978922176,
-15.8989996818882));
#70276=CARTESIAN_POINT('Ctrl Pts',(-18.6058615679212,-16.8388785369894,
-15.8987832045772));
#70277=CARTESIAN_POINT('Ctrl Pts',(-18.6140274945244,-16.8383971962887,
-15.8982866024987));
#70278=CARTESIAN_POINT('Ctrl Pts',(-18.6186261938086,-16.8381411830859,
-15.898006147527));
#70279=CARTESIAN_POINT('Ctrl Pts',(-18.6328371884397,-16.8373965570278,
-15.8971371162434));
#70280=CARTESIAN_POINT('Ctrl Pts',(-18.6424518513076,-16.8369584959363,
-15.8965458201374));
#70281=CARTESIAN_POINT('Ctrl Pts',(-18.7385993237839,-16.8332346561243,
-15.8906016737341));
#70282=CARTESIAN_POINT('Ctrl Pts',(-18.8252443275426,-16.8351961035337,
-15.8849958294741));
#70283=CARTESIAN_POINT('Ctrl Pts',(-19.0379889979674,-16.8530982102727,
-15.8709781822543));
#70284=CARTESIAN_POINT('Ctrl Pts',(-19.1632599948797,-16.8750942572814,
-15.8625168311259));
#70285=CARTESIAN_POINT('Ctrl Pts',(-19.3790109474436,-16.9333445130452,
-15.8480526332529));
#70286=CARTESIAN_POINT('Ctrl Pts',(-19.4703936016526,-16.9648567998986,
-15.8419579584493));
#70287=CARTESIAN_POINT('Ctrl Pts',(-19.5727827907089,-17.008203136903,-15.8351790325248));
#70288=CARTESIAN_POINT('Ctrl Pts',(-19.5861890734478,-17.0140431854904,
-15.834292273398));
#70289=CARTESIAN_POINT('Ctrl Pts',(-19.6065883488697,-17.0231821432437,
-15.8329440050806));
#70290=CARTESIAN_POINT('Ctrl Pts',(-19.6136253662043,-17.0263811465591,
-15.8324790915359));
#70291=CARTESIAN_POINT('Ctrl Pts',(-19.6264196572196,-17.03228215644,-15.8316341081777));
#70292=CARTESIAN_POINT('Ctrl Pts',(-19.6321825534869,-17.0349716889277,
-15.8312536145012));
#70293=CARTESIAN_POINT('Ctrl Pts',(-19.6446241860039,-17.0408465938407,
-15.830432357548));
#70294=CARTESIAN_POINT('Ctrl Pts',(-19.6512985338632,-17.0440411031908,
-15.829991916534));
#70295=CARTESIAN_POINT('Ctrl Pts',(-19.6694152820357,-17.0528292696567,
-15.8287966431054));
#70296=CARTESIAN_POINT('Ctrl Pts',(-19.6808242885097,-17.058491354599,-15.8280441983949));
#70297=CARTESIAN_POINT('Ctrl Pts',(-19.736864649105,-17.0869363407314,-15.8243486947409));
#70298=CARTESIAN_POINT('Ctrl Pts',(-19.7807305280544,-17.1111969848351,
-15.8214580021697));
#70299=CARTESIAN_POINT('Ctrl Pts',(-19.972520243798,-17.2263440055466,-15.8087586334641));
#70300=CARTESIAN_POINT('Ctrl Pts',(-20.1097822604082,-17.3336539136657,
-15.7995651478959));
#70301=CARTESIAN_POINT('Ctrl Pts',(-20.2767028774611,-17.5009007693087,
-15.7865789028613));
#70302=CARTESIAN_POINT('Ctrl Pts',(-20.3190029925107,-17.5472275947927,
-15.7830864138879));
#70303=CARTESIAN_POINT('Ctrl Pts',(-20.3790003013521,-17.6191011083125,
-15.777701159777));
#70304=CARTESIAN_POINT('Ctrl Pts',(-20.3982951698573,-17.6432728292479,
-15.7758951357452));
#70305=CARTESIAN_POINT('Ctrl Pts',(-20.4213765038163,-17.6735242089087,
-15.7736289639643));
#70306=CARTESIAN_POINT('Ctrl Pts',(-20.4256717692097,-17.6792131223155,
-15.7732025488737));
#70307=CARTESIAN_POINT('Ctrl Pts',(-20.4323832446634,-17.6881962007036,
-15.772528635461));
#70308=CARTESIAN_POINT('Ctrl Pts',(-20.43481883605,-17.6914759125037,-15.7722824692301));
#70309=CARTESIAN_POINT('Ctrl Pts',(-20.4393684433719,-17.6976395022762,
-15.7718195776586));
#70310=CARTESIAN_POINT('Ctrl Pts',(-20.4414846510287,-17.700521693468,-15.7716030085297));
#70311=CARTESIAN_POINT('Ctrl Pts',(-20.4463180500014,-17.7071396725437,
-15.7711054808261));
#70312=CARTESIAN_POINT('Ctrl Pts',(-20.4490303146206,-17.710878991301,-15.7708241874036));
#70313=CARTESIAN_POINT('Ctrl Pts',(-20.4573967018467,-17.7224932726025,
-15.7699500200099));
#70314=CARTESIAN_POINT('Ctrl Pts',(-20.4630088916803,-17.730398089008,-15.7693543805379));
#70315=CARTESIAN_POINT('Ctrl Pts',(-20.5258583273272,-17.8202227624746,
-15.7625810028211));
#70316=CARTESIAN_POINT('Ctrl Pts',(-20.5772738321383,-17.9060493234008,
-15.7560680765387));
#70317=CARTESIAN_POINT('Ctrl Pts',(-20.6995936513507,-18.1474645330186,
-15.7382365925715));
#70318=CARTESIAN_POINT('Ctrl Pts',(-20.7580649171488,-18.3085600868519,
-15.7269007381697));
#70319=CARTESIAN_POINT('Ctrl Pts',(-20.8065479299507,-18.5181762317816,
-15.7134188188318));
#70320=CARTESIAN_POINT('Ctrl Pts',(-20.8151860565393,-18.5617141470192,
-15.7106795887598));
#70321=CARTESIAN_POINT('Ctrl Pts',(-20.8243855588279,-18.6171611118075,
-15.7072652976819));
#70322=CARTESIAN_POINT('Ctrl Pts',(-20.8262235214717,-18.6288442934155,
-15.7065499894799));
#70323=CARTESIAN_POINT('Ctrl Pts',(-20.8290114871888,-18.6475880950504,
-15.7054088301419));
#70324=CARTESIAN_POINT('Ctrl Pts',(-20.8300239038325,-18.6546390479199,
-15.7049810097001));
#70325=CARTESIAN_POINT('Ctrl Pts',(-20.8318772341575,-18.6680264701936,
-15.7041714350991));
#70326=CARTESIAN_POINT('Ctrl Pts',(-20.832725073561,-18.6743618862296,-15.7037894660422));
#70327=CARTESIAN_POINT('Ctrl Pts',(-20.8345859301933,-18.6887627952022,
-15.7029237900794));
#70328=CARTESIAN_POINT('Ctrl Pts',(-20.835581216502,-18.6968305085283,-15.702440647848));
#70329=CARTESIAN_POINT('Ctrl Pts',(-20.8380346042422,-18.7177062736724,
-15.7011950975299));
#70330=CARTESIAN_POINT('Ctrl Pts',(-20.8394222483241,-18.7305223864685,
-15.7004349106064));
#70331=CARTESIAN_POINT('Ctrl Pts',(-20.8476032824,-18.8131247065847,-15.6955629343406));
#70332=CARTESIAN_POINT('Ctrl Pts',(-20.8510436183218,-18.8832033407658,
-15.6915582742407));
#70333=CARTESIAN_POINT('Ctrl Pts',(-20.8508787729878,-19.1457165811452,
-15.6768592876656));
#70334=CARTESIAN_POINT('Ctrl Pts',(-20.8245352123181,-19.3371656299188,
-15.6668249584927));
#70335=CARTESIAN_POINT('Ctrl Pts',(-20.7592947613957,-19.5703427201073,
-15.6531662356899));
#70336=CARTESIAN_POINT('Ctrl Pts',(-20.744197906492,-19.6177853425968,-15.6503027376871));
#70337=CARTESIAN_POINT('Ctrl Pts',(-20.7258385662826,-19.669140776792,-15.6470652387553));
#70338=CARTESIAN_POINT('Ctrl Pts',(-20.7242171427525,-19.6736283610162,
-15.6467811654567));
#70339=CARTESIAN_POINT('Ctrl Pts',(-20.7225805821192,-19.6781103693094,
-15.6464962362309));
#70340=CARTESIAN_POINT('Origin',(-18.734,-18.952,0.));
#70341=CARTESIAN_POINT('',(-20.7225805876025,-19.6781103542923,-14.843838552956));
#70342=CARTESIAN_POINT('',(-20.7193262595591,-19.6769292106295,-15.0663814047069));
#70343=CARTESIAN_POINT('',(-20.7225805821191,-19.6781103693095,0.));
#70344=CARTESIAN_POINT('',(-20.8523539179813,-18.9502594238256,-15.1109429533473));
#70345=CARTESIAN_POINT('Ctrl Pts',(-20.7193262595591,-19.6769292106295,
-15.0663814047069));
#70346=CARTESIAN_POINT('Ctrl Pts',(-20.8041091735384,-19.4439526196368,
-15.0812352542537));
#70347=CARTESIAN_POINT('Ctrl Pts',(-20.8501556558155,-19.196755797096,-15.0960891038005));
#70348=CARTESIAN_POINT('Ctrl Pts',(-20.8523539179813,-18.9502594238256,
-15.1109429533473));
#70349=CARTESIAN_POINT('Ctrl Pts',(-20.8509992391747,-18.95020519253,-15.1101643819126));
#70350=CARTESIAN_POINT('Ctrl Pts',(-20.8509308803988,-18.8695751088215,
-15.1145732053535));
#70351=CARTESIAN_POINT('Ctrl Pts',(-20.8462561257343,-18.7890199711534,
-15.1190367568054));
#70352=CARTESIAN_POINT('Ctrl Pts',(-20.8342751942077,-18.6853612765408,
-15.125069794828));
#70353=CARTESIAN_POINT('Ctrl Pts',(-20.8311546074106,-18.6618370303696,
-15.1264585298021));
#70354=CARTESIAN_POINT('Ctrl Pts',(-20.826756724514,-18.6324788069517,-15.1282217721656));
#70355=CARTESIAN_POINT('Ctrl Pts',(-20.8258491617714,-18.6265901302598,
-15.1285769647661));
#70356=CARTESIAN_POINT('Ctrl Pts',(-20.8242842195382,-18.6167132280723,
-15.1291753914717));
#70357=CARTESIAN_POINT('Ctrl Pts',(-20.8236402483669,-18.6127228718675,
-15.1294178945615));
#70358=CARTESIAN_POINT('Ctrl Pts',(-20.8224405319096,-18.6054218499359,
-15.1298629776525));
#70359=CARTESIAN_POINT('Ctrl Pts',(-20.821888330269,-18.6021106040616,-15.1300653585031));
#70360=CARTESIAN_POINT('Ctrl Pts',(-20.8207318336752,-18.595275969606,-15.1304841894194));
#70361=CARTESIAN_POINT('Ctrl Pts',(-20.8201264943957,-18.5917528234121,
-15.1307007002396));
#70362=CARTESIAN_POINT('Ctrl Pts',(-20.8187199420528,-18.5836889585382,
-15.1311976430554));
#70363=CARTESIAN_POINT('Ctrl Pts',(-20.8179128183668,-18.5791493267093,
-15.1314784069666));
#70364=CARTESIAN_POINT('Ctrl Pts',(-20.8153705427579,-18.5651165620324,
-15.1323493287048));
#70365=CARTESIAN_POINT('Ctrl Pts',(-20.8135853322361,-18.5556327855534,
-15.1329422231047));
#70366=CARTESIAN_POINT('Ctrl Pts',(-20.7945684717144,-18.4582737898767,
-15.1390707006034));
#70367=CARTESIAN_POINT('Ctrl Pts',(-20.7718442365237,-18.3715733301528,
-15.1448765239018));
#70368=CARTESIAN_POINT('Ctrl Pts',(-20.7294006552893,-18.2433845129372,
-15.1537504213448));
#70369=CARTESIAN_POINT('Ctrl Pts',(-20.7137086156514,-18.2006589367174,
-15.1567593942611));
#70370=CARTESIAN_POINT('Ctrl Pts',(-20.6822913302299,-18.1229537239433,
-15.1622977438439));
#70371=CARTESIAN_POINT('Ctrl Pts',(-20.6669687439335,-18.0878306009927,
-15.1648268511845));
#70372=CARTESIAN_POINT('Ctrl Pts',(-20.6103521144012,-17.9671027540647,
-15.1735853664));
#70373=CARTESIAN_POINT('Ctrl Pts',(-20.5642517997688,-17.883869940186,-15.1797341935906));
#70374=CARTESIAN_POINT('Ctrl Pts',(-20.4876366961899,-17.7651617441864,
-15.1886000796092));
#70375=CARTESIAN_POINT('Ctrl Pts',(-20.4612972481923,-17.7271443148118,
-15.1914568014498));
#70376=CARTESIAN_POINT('Ctrl Pts',(-20.426585568463,-17.6803920348148,-15.1949948796788));
#70377=CARTESIAN_POINT('Ctrl Pts',(-20.419357268767,-17.6708272522518,-15.1957201083331));
#70378=CARTESIAN_POINT('Ctrl Pts',(-20.4076833152254,-17.6556495796288,
-15.1968733115488));
#70379=CARTESIAN_POINT('Ctrl Pts',(-20.4032898418012,-17.6499970514318,
-15.1973033293901));
#70380=CARTESIAN_POINT('Ctrl Pts',(-20.3949236797005,-17.6393453227619,
-15.198114728903));
#70381=CARTESIAN_POINT('Ctrl Pts',(-20.390956890882,-17.6343416092918,-15.1984963387046));
#70382=CARTESIAN_POINT('Ctrl Pts',(-20.3819269075974,-17.6230564354904,
-15.1993580712028));
#70383=CARTESIAN_POINT('Ctrl Pts',(-20.3768503032154,-17.6167857945579,
-15.1998376492528));
#70384=CARTESIAN_POINT('Ctrl Pts',(-20.3617628824936,-17.5983660731065,
-15.2012487479317));
#70385=CARTESIAN_POINT('Ctrl Pts',(-20.351652125249,-17.5862992892667,-15.2021762150453));
#70386=CARTESIAN_POINT('Ctrl Pts',(-20.2604784484587,-17.4799204241743,
-15.2103833193024));
#70387=CARTESIAN_POINT('Ctrl Pts',(-20.1713821987607,-17.3928036884123,
-15.2173013409388));
#70388=CARTESIAN_POINT('Ctrl Pts',(-19.9454701124689,-17.2078337596716,
-15.2332484884381));
#70389=CARTESIAN_POINT('Ctrl Pts',(-19.8036698529555,-17.1174519136689,
-15.2421094361227));
#70390=CARTESIAN_POINT('Ctrl Pts',(-19.6396557105219,-17.0384464582166,
-15.2526982253465));
#70391=CARTESIAN_POINT('Ctrl Pts',(-19.6265229277816,-17.0322859007933,
-15.2535485548977));
#70392=CARTESIAN_POINT('Ctrl Pts',(-19.6037124115813,-17.0218701949354,
-15.2550315091401));
#70393=CARTESIAN_POINT('Ctrl Pts',(-19.5940640423333,-17.01755160938,-15.2556606039237));
#70394=CARTESIAN_POINT('Ctrl Pts',(-19.5800043974146,-17.011384522754,-15.2565805517638));
#70395=CARTESIAN_POINT('Ctrl Pts',(-19.5756183861498,-17.0094783496594,
-15.2568679898402));
#70396=CARTESIAN_POINT('Ctrl Pts',(-19.5679101949997,-17.0061593539945,
-15.2573740060357));
#70397=CARTESIAN_POINT('Ctrl Pts',(-19.5645907650565,-17.0047401267838,
-15.2575921945907));
#70398=CARTESIAN_POINT('Ctrl Pts',(-19.5576346682157,-17.0017870600549,
-15.2580500336323));
#70399=CARTESIAN_POINT('Ctrl Pts',(-19.553997350716,-17.0002549034147,-15.2582897793109));
#70400=CARTESIAN_POINT('Ctrl Pts',(-19.5443530978565,-16.9962241479842,
-15.2589263254252));
#70401=CARTESIAN_POINT('Ctrl Pts',(-19.538338948178,-16.9937430759912,-15.2593241632859));
#70402=CARTESIAN_POINT('Ctrl Pts',(-19.5128391712561,-16.9833607066627,
-15.2610144377901));
#70403=CARTESIAN_POINT('Ctrl Pts',(-19.4932485805838,-16.9757225302507,
-15.2623215259099));
#70404=CARTESIAN_POINT('Ctrl Pts',(-19.4671271787103,-16.9659837607493,
-15.2640725150997));
#70405=CARTESIAN_POINT('Ctrl Pts',(-19.4606944937141,-16.9636209935828,
-15.2645043668025));
#70406=CARTESIAN_POINT('Ctrl Pts',(-19.2917024445415,-16.9024786952497,
-15.2758644884146));
#70407=CARTESIAN_POINT('Ctrl Pts',(-19.1225682382837,-16.8637987004395,
-15.2875343842416));
#70408=CARTESIAN_POINT('Ctrl Pts',(-18.8418510692378,-16.8349237650268,
-15.3059395948085));
#70409=CARTESIAN_POINT('Ctrl Pts',(-18.7323719107138,-16.8321775126924,
-15.3128999613875));
#70410=CARTESIAN_POINT('Ctrl Pts',(-18.6051508991758,-16.83884786069,-15.3206977000676));
#70411=CARTESIAN_POINT('Ctrl Pts',(-18.587158732243,-16.8400218447377,-15.3217940493735));
#70412=CARTESIAN_POINT('Ctrl Pts',(-18.5607995007167,-16.8420802612564,
-15.3233911888492));
#70413=CARTESIAN_POINT('Ctrl Pts',(-18.552419574071,-16.8427849163734,-15.3238975964283));
#70414=CARTESIAN_POINT('Ctrl Pts',(-18.5376422210812,-16.8441162418849,
-15.3247883008332));
#70415=CARTESIAN_POINT('Ctrl Pts',(-18.5312430750704,-16.8447221479184,
-15.325173245206));
#70416=CARTESIAN_POINT('Ctrl Pts',(-18.5187537019778,-16.8459621270846,
-15.3259230945478));
#70417=CARTESIAN_POINT('Ctrl Pts',(-18.5126632759386,-16.8465934960775,
-15.3262880805584));
#70418=CARTESIAN_POINT('Ctrl Pts',(-18.4962625038533,-16.8483656484066,
-15.327269165779));
#70419=CARTESIAN_POINT('Ctrl Pts',(-18.4859575765167,-16.8495558118618,
-15.3278837058512));
#70420=CARTESIAN_POINT('Ctrl Pts',(-18.447709328535,-16.854258405811,-15.330157970957));
#70421=CARTESIAN_POINT('Ctrl Pts',(-18.419827439645,-16.858252675877,-15.3318025101184));
#70422=CARTESIAN_POINT('Ctrl Pts',(-18.3853154434712,-16.8639017244639,
-15.3338244722909));
#70423=CARTESIAN_POINT('Ctrl Pts',(-18.378603634609,-16.8650336003671,-15.3342170583226));
#70424=CARTESIAN_POINT('Ctrl Pts',(-18.1687040477466,-16.9014729129972,
-15.3464756590207));
#70425=CARTESIAN_POINT('Ctrl Pts',(-17.9717746191708,-16.9662432872382,
-15.3572865048384));
#70426=CARTESIAN_POINT('Ctrl Pts',(-17.7393115003368,-17.0824640721618,
-15.3716602622996));
#70427=CARTESIAN_POINT('Ctrl Pts',(-17.6922372995949,-17.1082810729171,
-15.3746717993785));
#70428=CARTESIAN_POINT('Ctrl Pts',(-17.6222407070437,-17.1502064063392,
-15.3793812548432));
#70429=CARTESIAN_POINT('Ctrl Pts',(-17.5985707045904,-17.1650279731896,
-15.3810160152549));
#70430=CARTESIAN_POINT('Ctrl Pts',(-17.5694284467914,-17.1840888898497,
-15.3830909759209));
#70431=CARTESIAN_POINT('Ctrl Pts',(-17.5636733720524,-17.1878933771279,
-15.3835038308042));
#70432=CARTESIAN_POINT('Ctrl Pts',(-17.5545824903361,-17.1939671179346,
-15.3841610694151));
#70433=CARTESIAN_POINT('Ctrl Pts',(-17.5512343397524,-17.1962179324193,
-15.3844042289519));
#70434=CARTESIAN_POINT('Ctrl Pts',(-17.5449227304335,-17.2004871957905,
-15.384864732702));
#70435=CARTESIAN_POINT('Ctrl Pts',(-17.5419579582829,-17.2025036077876,
-15.3850819401012));
#70436=CARTESIAN_POINT('Ctrl Pts',(-17.535179518464,-17.2071390151867,-15.3855805833949));
#70437=CARTESIAN_POINT('Ctrl Pts',(-17.531369307363,-17.209762984131,-15.3858623543444));
#70438=CARTESIAN_POINT('Ctrl Pts',(-17.5212520442076,-17.2167794178452,
-15.3866144216391));
#70439=CARTESIAN_POINT('Ctrl Pts',(-17.514960327722,-17.2211937294096,-15.3870861499966));
#70440=CARTESIAN_POINT('Ctrl Pts',(-17.4703777093284,-17.2528368781108,
-15.3904567642226));
#70441=CARTESIAN_POINT('Ctrl Pts',(-17.4329815702175,-17.2812974782625,
-15.3934314401874));
#70442=CARTESIAN_POINT('Ctrl Pts',(-17.3833349080328,-17.3217594753665,
-15.3975525970894));
#70443=CARTESIAN_POINT('Ctrl Pts',(-17.3702346136542,-17.332702527244,-15.3986571806867));
#70444=CARTESIAN_POINT('Ctrl Pts',(-17.2464260212764,-17.4386915067362,
-15.4092511989913));
#70445=CARTESIAN_POINT('Ctrl Pts',(-17.1456888572926,-17.5447863119784,
-15.4190325569378));
#70446=CARTESIAN_POINT('Ctrl Pts',(-16.9946655190774,-17.7409138466012,
-15.4350922951708));
#70447=CARTESIAN_POINT('Ctrl Pts',(-16.9385411023579,-17.8257910000771,
-15.4415203306821));
#70448=CARTESIAN_POINT('Ctrl Pts',(-16.88148535309,-17.9272577741716,-15.4486188870818));
#70449=CARTESIAN_POINT('Ctrl Pts',(-16.8743809509526,-17.9402074539809,
-15.4495146969995));
#70450=CARTESIAN_POINT('Ctrl Pts',(-16.8637510909029,-17.9600734666077,
-15.4508738179381));
#70451=CARTESIAN_POINT('Ctrl Pts',(-16.8601272900813,-17.9669363984239,
-15.4513406184065));
#70452=CARTESIAN_POINT('Ctrl Pts',(-16.8536021175323,-17.979460404038,-15.4521875853037));
#70453=CARTESIAN_POINT('Ctrl Pts',(-16.8506883782703,-17.9851148987971,
-15.4525681857889));
#70454=CARTESIAN_POINT('Ctrl Pts',(-16.8444520088777,-17.9973525441892,
-15.4533880584895));
#70455=CARTESIAN_POINT('Ctrl Pts',(-16.8411381918925,-18.0039401109855,
-15.4538270171722));
#70456=CARTESIAN_POINT('Ctrl Pts',(-16.8322437831059,-18.0218539287416,
-15.4550143367789));
#70457=CARTESIAN_POINT('Ctrl Pts',(-16.8267299339704,-18.0332131215612,
-15.4557603635027));
#70458=CARTESIAN_POINT('Ctrl Pts',(-16.8003761900956,-18.0887647062782,
-15.4593764127651));
#70459=CARTESIAN_POINT('Ctrl Pts',(-16.7809678607989,-18.1336222051621,
-15.4621967943453));
#70460=CARTESIAN_POINT('Ctrl Pts',(-16.754904355692,-18.2000845599324,-15.4662533971502));
#70461=CARTESIAN_POINT('Ctrl Pts',(-16.7470156733704,-18.2211855716913,
-15.467523885315));
#70462=CARTESIAN_POINT('Ctrl Pts',(-16.6860209092723,-18.3926310620439,
-15.4777214838548));
#70463=CARTESIAN_POINT('Ctrl Pts',(-16.649720985206,-18.5484019781177,-15.4861694750401));
#70464=CARTESIAN_POINT('Ctrl Pts',(-16.6245782312839,-18.7639904758771,
-15.4981383683942));
#70465=CARTESIAN_POINT('Ctrl Pts',(-16.6202438299625,-18.8214561593737,
-15.5013600872869));
#70466=CARTESIAN_POINT('Ctrl Pts',(-16.6172493382223,-18.9082717148673,
-15.5063661736089));
#70467=CARTESIAN_POINT('Ctrl Pts',(-16.6168471589145,-18.9375369349987,
-15.5080775254896));
#70468=CARTESIAN_POINT('Ctrl Pts',(-16.6171006974187,-18.9738038432122,
-15.5102380946414));
#70469=CARTESIAN_POINT('Ctrl Pts',(-16.6171844278859,-18.9808079047586,
-15.5106571949296));
#70470=CARTESIAN_POINT('Ctrl Pts',(-16.6173715576251,-18.9918685717879,
-15.5113221149092));
#70471=CARTESIAN_POINT('Ctrl Pts',(-16.6174518649233,-18.9959255888242,
-15.5115666611924));
#70472=CARTESIAN_POINT('Ctrl Pts',(-16.6176249921721,-19.0035620746099,
-15.5120282446984));
#70473=CARTESIAN_POINT('Ctrl Pts',(-16.6177152293857,-19.0071415474771,
-15.5122451360844));
#70474=CARTESIAN_POINT('Ctrl Pts',(-16.6179417807768,-19.0153060330385,
-15.5127410489168));
#70475=CARTESIAN_POINT('Ctrl Pts',(-16.6180839160088,-19.019890835571,-15.5130203922669));
#70476=CARTESIAN_POINT('Ctrl Pts',(-16.618499507527,-19.0320231629289,-15.5137618067763));
#70477=CARTESIAN_POINT('Ctrl Pts',(-16.6187984518493,-19.0395696697087,
-15.5142252477047));
#70478=CARTESIAN_POINT('Ctrl Pts',(-16.6211260833301,-19.0913244605158,
-15.5174183993767));
#70479=CARTESIAN_POINT('Ctrl Pts',(-16.624500053329,-19.1354580090972,-15.520215388163));
#70480=CARTESIAN_POINT('Ctrl Pts',(-16.6305885528259,-19.191799023117,-15.52385438502));
#70481=CARTESIAN_POINT('Ctrl Pts',(-16.6320317279074,-19.2041361943857,
-15.524655459839));
#70482=CARTESIAN_POINT('Ctrl Pts',(-16.6545170514119,-19.382721211433,-15.536306501986));
#70483=CARTESIAN_POINT('Ctrl Pts',(-16.6951167656538,-19.5459131751443,
-15.547585407901));
#70484=CARTESIAN_POINT('Ctrl Pts',(-16.7753276157099,-19.7574367102437,
-15.5621666260113));
#70485=CARTESIAN_POINT('Ctrl Pts',(-16.7983831848399,-19.8113685614429,
-15.5658877801012));
#70486=CARTESIAN_POINT('Ctrl Pts',(-16.8391093525476,-19.8966509727386,
-15.5717699087376));
#70487=CARTESIAN_POINT('Ctrl Pts',(-16.8553900987904,-19.9286274173903,
-15.5739751542906));
#70488=CARTESIAN_POINT('Ctrl Pts',(-16.8777080193095,-19.9698358211046,
-15.5768185415365));
#70489=CARTESIAN_POINT('Ctrl Pts',(-16.8830147061486,-19.9794546828792,
-15.5774823643719));
#70490=CARTESIAN_POINT('Ctrl Pts',(-16.891794215331,-19.9950795596287,-15.578560995279));
#70491=CARTESIAN_POINT('Ctrl Pts',(-16.8952220621483,-20.0011104888595,
-15.5789774061524));
#70492=CARTESIAN_POINT('Ctrl Pts',(-16.901890227451,-20.0127093287419,-15.5797784521697));
#70493=CARTESIAN_POINT('Ctrl Pts',(-16.9051264339512,-20.0182795034951,
-15.5801632298342));
#70494=CARTESIAN_POINT('Ctrl Pts',(-16.9126218844305,-20.0310461939897,
-15.5810453753683));
#70495=CARTESIAN_POINT('Ctrl Pts',(-16.9168984619197,-20.0382324484232,
-15.5815421073966));
#70496=CARTESIAN_POINT('Ctrl Pts',(-16.9284341611487,-20.057357967057,-15.5828647225167));
#70497=CARTESIAN_POINT('Ctrl Pts',(-16.9357691690271,-20.0692511473504,
-15.5836878278341));
#70498=CARTESIAN_POINT('Ctrl Pts',(-16.9966065026245,-20.1657430266225,
-15.5903731984827));
#70499=CARTESIAN_POINT('Ctrl Pts',(-17.055932749397,-20.2465278285754,-15.5960081273972));
#70500=CARTESIAN_POINT('Ctrl Pts',(-17.2320281650651,-20.4537645666326,
-15.6109932072816));
#70501=CARTESIAN_POINT('Ctrl Pts',(-17.3588112912004,-20.5706601199029,
-15.6200250113701));
#70502=CARTESIAN_POINT('Ctrl Pts',(-17.5307321932079,-20.6942485935035,
-15.6320880332919));
#70503=CARTESIAN_POINT('Ctrl Pts',(-17.5638065631404,-20.7166332288957,
-15.6344039137322));
#70504=CARTESIAN_POINT('Ctrl Pts',(-17.6039778686457,-20.7421949865848,
-15.6372361337777));
#70505=CARTESIAN_POINT('Ctrl Pts',(-17.6104865023576,-20.7462869123569,
-15.6376956093319));
#70506=CARTESIAN_POINT('Ctrl Pts',(-17.6205913264878,-20.7525631976271,
-15.6384101064369));
#70507=CARTESIAN_POINT('Ctrl Pts',(-17.6241720607498,-20.7547724890996,
-15.6386635165676));
#70508=CARTESIAN_POINT('Ctrl Pts',(-17.6307962253214,-20.7588323438168,
-15.6391327660087));
#70509=CARTESIAN_POINT('Ctrl Pts',(-17.6338377493117,-20.7606859065998,
-15.6393484044117));
#70510=CARTESIAN_POINT('Ctrl Pts',(-17.6406882381524,-20.7648370523335,
-15.639834492338));
#70511=CARTESIAN_POINT('Ctrl Pts',(-17.6444997500179,-20.7671302959734,
-15.6401052179113));
#70512=CARTESIAN_POINT('Ctrl Pts',(-17.6542698666072,-20.7729667483636,
-15.6407998143986));
#70513=CARTESIAN_POINT('Ctrl Pts',(-17.660238646548,-20.7764927000111,-15.641224765878));
#70514=CARTESIAN_POINT('Ctrl Pts',(-17.6951896539675,-20.7969084812697,
-15.643716171218));
#70515=CARTESIAN_POINT('Ctrl Pts',(-17.7245509896218,-20.8131358476201,
-15.6458212515246));
#70516=CARTESIAN_POINT('Ctrl Pts',(-17.7704989558741,-20.8371231642198,
-15.6491198083931));
#70517=CARTESIAN_POINT('Ctrl Pts',(-17.7868230982952,-20.8453777982325,
-15.6502925267748));
#70518=CARTESIAN_POINT('Ctrl Pts',(-17.8254385472691,-20.864280129405,-15.6530652774896));
#70519=CARTESIAN_POINT('Ctrl Pts',(-17.8478131982875,-20.8747511780483,
-15.6546708074526));
#70520=CARTESIAN_POINT('Ctrl Pts',(-17.9113760340621,-20.9031526032054,
-15.6592198089));
#70521=CARTESIAN_POINT('Ctrl Pts',(-17.9529587003891,-20.920166908421,-15.6621815075243));
#70522=CARTESIAN_POINT('Ctrl Pts',(-18.097517025324,-20.9740125240048,-15.6723716441283));
#70523=CARTESIAN_POINT('Ctrl Pts',(-18.2027950753033,-21.0041866433303,
-15.6796016753953));
#70524=CARTESIAN_POINT('Ctrl Pts',(-18.3638784998297,-21.0371211412524,
-15.690169510304));
#70525=CARTESIAN_POINT('Ctrl Pts',(-18.4182310026962,-21.046041751751,-15.6936557104331));
#70526=CARTESIAN_POINT('Ctrl Pts',(-18.5068944925558,-21.0570623285956,
-15.6992091499861));
#70527=CARTESIAN_POINT('Ctrl Pts',(-18.5410147599938,-21.0604641879492,
-15.7013147569704));
#70528=CARTESIAN_POINT('Ctrl Pts',(-18.5859799086462,-21.0638465438054,
-15.7040499146466));
#70529=CARTESIAN_POINT('Ctrl Pts',(-18.5967617771021,-21.0645746019926,
-15.704702777422));
#70530=CARTESIAN_POINT('Ctrl Pts',(-18.6144340912719,-21.065632079852,-15.705768105147));
#70531=CARTESIAN_POINT('Ctrl Pts',(-18.6213213107339,-21.0660104281309,
-15.7061820985873));
#70532=CARTESIAN_POINT('Ctrl Pts',(-18.6346591962457,-21.0666777761213,
-15.7069815944132));
#70533=CARTESIAN_POINT('Ctrl Pts',(-18.6411095689086,-21.0669709362895,
-15.7073672229278));
#70534=CARTESIAN_POINT('Ctrl Pts',(-18.6560100703333,-21.0675798431756,
-15.7082557285045));
#70535=CARTESIAN_POINT('Ctrl Pts',(-18.6644609875387,-21.0678744837279,
-15.7087579390911));
#70536=CARTESIAN_POINT('Ctrl Pts',(-18.6872016704759,-21.0685309440704,
-15.7101048746185));
#70537=CARTESIAN_POINT('Ctrl Pts',(-18.7014938661136,-21.0687986883588,
-15.7109466558997));
#70538=CARTESIAN_POINT('Ctrl Pts',(-18.8329520578782,-21.069929634311,-15.7186481553049));
#70539=CARTESIAN_POINT('Ctrl Pts',(-18.9500047372853,-21.0612094951556,
-15.7251892443868));
#70540=CARTESIAN_POINT('Ctrl Pts',(-19.2275945879108,-21.0171651695816,
-15.7405741597957));
#70541=CARTESIAN_POINT('Ctrl Pts',(-19.3858917006964,-20.9727839205466,
-15.7492315713575));
#70542=CARTESIAN_POINT('Ctrl Pts',(-19.566331432673,-20.8987631448044,-15.7604463711599));
#70543=CARTESIAN_POINT('Ctrl Pts',(-19.5949287816643,-20.8862863686575,
-15.7622678969541));
#70544=CARTESIAN_POINT('Ctrl Pts',(-19.6297250679824,-20.870180569253,-15.7645513400857));
#70545=CARTESIAN_POINT('Ctrl Pts',(-19.636196528423,-20.8671452985234,-15.7649789126623));
#70546=CARTESIAN_POINT('Ctrl Pts',(-19.6463460496562,-20.8623220696694,
-15.7656542488097));
#70547=CARTESIAN_POINT('Ctrl Pts',(-19.6500345816461,-20.8605560952633,
-15.7659006709));
#70548=CARTESIAN_POINT('Ctrl Pts',(-19.6569379597282,-20.8572263128842,
-15.7663637733777));
#70549=CARTESIAN_POINT('Ctrl Pts',(-19.6601539694199,-20.8556650453968,
-15.7665802959298));
#70550=CARTESIAN_POINT('Ctrl Pts',(-19.6675103568105,-20.8520707065325,
-15.7670773572291));
#70551=CARTESIAN_POINT('Ctrl Pts',(-19.6716480424145,-20.850032250443,-15.7673582284861));
#70552=CARTESIAN_POINT('Ctrl Pts',(-19.6824717760563,-20.8446558418092,
-15.7680962857257));
#70553=CARTESIAN_POINT('Ctrl Pts',(-19.6891468016376,-20.8412960141394,
-15.768554787734));
#70554=CARTESIAN_POINT('Ctrl Pts',(-19.7338274804456,-20.8185090032766,
-15.771645636902));
#70555=CARTESIAN_POINT('Ctrl Pts',(-19.7712531445933,-20.7979729673008,
-15.7743405811426));
#70556=CARTESIAN_POINT('Ctrl Pts',(-19.8142369072539,-20.7726672157876,
-15.7775397000198));
#70557=CARTESIAN_POINT('Ctrl Pts',(-19.8204255206058,-20.7689811425854,
-15.7780028777329));
#70558=CARTESIAN_POINT('Ctrl Pts',(-19.9612667917299,-20.6841162126135,
-15.7886011420379));
#70559=CARTESIAN_POINT('Ctrl Pts',(-20.086479597217,-20.5882189962405,-15.7991743953588));
#70560=CARTESIAN_POINT('Ctrl Pts',(-20.2683631254329,-20.4136489942513,
-15.8155535235058));
#70561=CARTESIAN_POINT('Ctrl Pts',(-20.3323175777072,-20.3434284351539,
-15.8215791495485));
#70562=CARTESIAN_POINT('Ctrl Pts',(-20.4046232472794,-20.2524468092857,
-15.8287172278721));
#70563=CARTESIAN_POINT('Ctrl Pts',(-20.4176410443256,-20.2355485282016,
-15.8300172747308));
#70564=CARTESIAN_POINT('Ctrl Pts',(-20.4357852640571,-20.2112445758436,
-15.8318515008308));
#70565=CARTESIAN_POINT('Ctrl Pts',(-20.4411229329346,-20.2039989147406,
-15.8323939340964));
#70566=CARTESIAN_POINT('Ctrl Pts',(-20.4502504309102,-20.191441820576,-15.8333265210172));
#70567=CARTESIAN_POINT('Ctrl Pts',(-20.4540621746829,-20.186146541095,-15.8337175219323));
#70568=CARTESIAN_POINT('Ctrl Pts',(-20.4613129493773,-20.1759749093206,
-15.8344643000007));
#70569=CARTESIAN_POINT('Ctrl Pts',(-20.4647559571994,-20.1711014812041,
-15.834820227979));
#70570=CARTESIAN_POINT('Ctrl Pts',(-20.4736538365658,-20.1583932471106,
-15.8357435658547));
#70571=CARTESIAN_POINT('Ctrl Pts',(-20.4790764370083,-20.1505359282427,
-15.8363097396569));
#70572=CARTESIAN_POINT('Ctrl Pts',(-20.4973780544504,-20.123629447374,-15.8382327969975));
#70573=CARTESIAN_POINT('Ctrl Pts',(-20.5100000716278,-20.1044068428274,
-15.8395799884682));
#70574=CARTESIAN_POINT('Ctrl Pts',(-20.6034752477959,-19.9568649445858,
-15.849729202511));
#70575=CARTESIAN_POINT('Ctrl Pts',(-20.6706038316627,-19.8204578153052,
-15.857987109407));
#70576=CARTESIAN_POINT('Ctrl Pts',(-20.7225805818996,-19.6781103699108,
-15.8662165012922));
#70577=CARTESIAN_POINT('',(-20.850999748114,-18.9530327076519,-14.890777192852));
#70578=CARTESIAN_POINT('Ctrl Pts',(-20.7225805821192,-19.6781103693094,
-15.6464962362309));
#70579=CARTESIAN_POINT('Ctrl Pts',(-20.7215382005989,-19.6809651139018,
-15.6463147550481));
#70580=CARTESIAN_POINT('Ctrl Pts',(-20.7204896781789,-19.6838175964211,
-15.6461329266281));
#70581=CARTESIAN_POINT('Ctrl Pts',(-20.7178168237568,-19.6910409683998,
-15.6456712114951));
#70582=CARTESIAN_POINT('Ctrl Pts',(-20.7161841986203,-19.6954087334581,
-15.6453908458301));
#70583=CARTESIAN_POINT('Ctrl Pts',(-20.713268966459,-19.703129981681,-15.6448930705602));
#70584=CARTESIAN_POINT('Ctrl Pts',(-20.711992242547,-19.7064856388513,-15.644676014502));
#70585=CARTESIAN_POINT('Ctrl Pts',(-20.7092701408642,-19.7135858327957,
-15.6442151944605));
#70586=CARTESIAN_POINT('Ctrl Pts',(-20.707822671301,-19.7173294530747,-15.6439713114886));
#70587=CARTESIAN_POINT('Ctrl Pts',(-20.7038921043828,-19.727409838564,-15.6433121929136));
#70588=CARTESIAN_POINT('Ctrl Pts',(-20.7013891053025,-19.7337387198285,
-15.6428957881994));
#70589=CARTESIAN_POINT('Ctrl Pts',(-20.6888792590765,-19.7649294771773,
-15.6408312283235));
#70590=CARTESIAN_POINT('Ctrl Pts',(-20.6784319306481,-19.7896106279086,
-15.6391586007787));
#70591=CARTESIAN_POINT('Ctrl Pts',(-20.6469617777437,-19.8601931391508,
-15.6342757408071));
#70592=CARTESIAN_POINT('Ctrl Pts',(-20.624762662322,-19.9055478045807,-15.6310149021864));
#70593=CARTESIAN_POINT('Ctrl Pts',(-20.5384183300512,-20.0670626330061,
-15.6190523714896));
#70594=CARTESIAN_POINT('Ctrl Pts',(-20.465010723893,-20.1779261629286,-15.6101841681029));
#70595=CARTESIAN_POINT('Ctrl Pts',(-20.3168837375819,-20.3615484045732,
-15.5948582422368));
#70596=CARTESIAN_POINT('Ctrl Pts',(-20.2462642317458,-20.4370622909368,
-15.5883172978543));
#70597=CARTESIAN_POINT('Ctrl Pts',(-20.1600892169511,-20.5166583489903,
-15.5811566450355));
#70598=CARTESIAN_POINT('Ctrl Pts',(-20.1496786630315,-20.5260839055539,
-15.5803038367314));
#70599=CARTESIAN_POINT('Ctrl Pts',(-20.1329049467825,-20.5409695473105,
-15.5789489441957));
#70600=CARTESIAN_POINT('Ctrl Pts',(-20.1266019392175,-20.546496508136,-15.5784440592285));
#70601=CARTESIAN_POINT('Ctrl Pts',(-20.1153950606441,-20.5562064165061,
-15.5775537585517));
#70602=CARTESIAN_POINT('Ctrl Pts',(-20.1105046347987,-20.5604046543496,
-15.5771677101394));
#70603=CARTESIAN_POINT('Ctrl Pts',(-20.1003178022324,-20.5690691576568,
-15.5763686079997));
#70604=CARTESIAN_POINT('Ctrl Pts',(-20.0950184846581,-20.5735318940789,
-15.5759557021595));
#70605=CARTESIAN_POINT('Ctrl Pts',(-20.0812910645662,-20.5849775189835,
-15.5748932258545));
#70606=CARTESIAN_POINT('Ctrl Pts',(-20.0728304786987,-20.5919212622195,
-15.5742452531959));
#70607=CARTESIAN_POINT('Ctrl Pts',(-20.0366931772938,-20.6211136748238,
-15.5715060498402));
#70608=CARTESIAN_POINT('Ctrl Pts',(-20.0085118919996,-20.6427305013262,
-15.5694401576718));
#70609=CARTESIAN_POINT('Ctrl Pts',(-19.9330683626312,-20.6976416156175,
-15.5640773526727));
#70610=CARTESIAN_POINT('Ctrl Pts',(-19.8849624425687,-20.7297276991296,
-15.5608243703641));
#70611=CARTESIAN_POINT('Ctrl Pts',(-19.6972067777359,-20.8441380470949,
-15.548624870114));
#70612=CARTESIAN_POINT('Ctrl Pts',(-19.549598286454,-20.9122927572047,-15.5400738501042));
#70613=CARTESIAN_POINT('Ctrl Pts',(-19.3750795392248,-20.9697155083056,
-15.5298130487453));
#70614=CARTESIAN_POINT('Ctrl Pts',(-19.3543872166229,-20.9761735346412,
-15.5285934138505));
#70615=CARTESIAN_POINT('Ctrl Pts',(-19.293322846051,-20.9942073073806,-15.5249757427993));
#70616=CARTESIAN_POINT('Ctrl Pts',(-19.2527036715844,-21.0049000715263,
-15.5225458747638));
#70617=CARTESIAN_POINT('Ctrl Pts',(-19.2045512407733,-21.0160556781879,
-15.5196092950154));
#70618=CARTESIAN_POINT('Ctrl Pts',(-19.197297201433,-21.0176960115941,-15.5191654218524));
#70619=CARTESIAN_POINT('Ctrl Pts',(-19.18554097764,-21.02028937109,-15.518443438665));
#70620=CARTESIAN_POINT('Ctrl Pts',(-19.181043993016,-21.0212660158721,-15.5181666465004));
#70621=CARTESIAN_POINT('Ctrl Pts',(-19.1730489573006,-21.0229750809553,
-15.5176733897125));
#70622=CARTESIAN_POINT('Ctrl Pts',(-19.1695521994188,-21.023713313711,-15.5174572611286));
#70623=CARTESIAN_POINT('Ctrl Pts',(-19.1620433600095,-21.0252787228024,
-15.5169922892256));
#70624=CARTESIAN_POINT('Ctrl Pts',(-19.1580308018883,-21.0261030974535,
-15.5167432954317));
#70625=CARTESIAN_POINT('Ctrl Pts',(-19.1469794525936,-21.0283401725998,
-15.5160561283976));
#70626=CARTESIAN_POINT('Ctrl Pts',(-19.1399359049353,-21.0297287066164,
-15.5156166134304));
#70627=CARTESIAN_POINT('Ctrl Pts',(-19.1018144991776,-21.0370425511314,
-15.5132299795146));
#70628=CARTESIAN_POINT('Ctrl Pts',(-19.0706156026954,-21.0423061099051,
-15.5112485289031));
#70629=CARTESIAN_POINT('Ctrl Pts',(-18.8775501419016,-21.0704440605135,
-15.4988613725745));
#70630=CARTESIAN_POINT('Ctrl Pts',(-18.7136063234049,-21.0752041327929,
-15.4878510547611));
#70631=CARTESIAN_POINT('Ctrl Pts',(-18.4341378647768,-21.0509217587739,
-15.4695259740205));
#70632=CARTESIAN_POINT('Ctrl Pts',(-18.3185533404816,-21.0311348620421,
-15.4620692031308));
#70633=CARTESIAN_POINT('Ctrl Pts',(-18.1913415565047,-20.9983174456796,
-15.4540473203771));
#70634=CARTESIAN_POINT('Ctrl Pts',(-18.1775384304006,-20.9946071115307,
-15.4531791517874));
#70635=CARTESIAN_POINT('Ctrl Pts',(-18.155630753867,-20.988479685448,-15.4518045969395));
#70636=CARTESIAN_POINT('Ctrl Pts',(-18.1475014682284,-20.9861533790708,
-15.4512952809801));
#70637=CARTESIAN_POINT('Ctrl Pts',(-18.1331893047511,-20.9819648271838,
-15.450399838472));
#70638=CARTESIAN_POINT('Ctrl Pts',(-18.1270006416119,-20.9801228935837,
-15.4500130554991));
#70639=CARTESIAN_POINT('Ctrl Pts',(-18.1142184360722,-20.9762547742637,
-15.4492149990802));
#70640=CARTESIAN_POINT('Ctrl Pts',(-18.1076261681221,-20.9742246172432,
-15.4488038608594));
#70641=CARTESIAN_POINT('Ctrl Pts',(-18.0907312497104,-20.9689311107601,
-15.4477512714696));
#70642=CARTESIAN_POINT('Ctrl Pts',(-18.0804433716501,-20.9656209997779,
-15.4471113609103));
#70643=CARTESIAN_POINT('Ctrl Pts',(-18.0376200206075,-20.9514798733221,
-15.4444516501353));
#70644=CARTESIAN_POINT('Ctrl Pts',(-18.0053236990031,-20.9399375956609,
-15.4424553571148));
#70645=CARTESIAN_POINT('Ctrl Pts',(-17.9219259782214,-20.9078266242942,
-15.4373139163172));
#70646=CARTESIAN_POINT('Ctrl Pts',(-17.8713207626631,-20.8860390841569,
-15.4342081046017));
#70647=CARTESIAN_POINT('Ctrl Pts',(-17.7229740603503,-20.8151871403612,
-15.4250667425354));
#70648=CARTESIAN_POINT('Ctrl Pts',(-17.6281230726459,-20.760501279765,-15.4191799316769));
#70649=CARTESIAN_POINT('Ctrl Pts',(-17.5024545718971,-20.674449547118,-15.4108878219961));
#70650=CARTESIAN_POINT('Ctrl Pts',(-17.4677376394491,-20.649090459584,-15.4085381838538));
#70651=CARTESIAN_POINT('Ctrl Pts',(-17.3741929581124,-20.5762912399506,
-15.4019762949796));
#70652=CARTESIAN_POINT('Ctrl Pts',(-17.3171014990814,-20.5267359424784,
-15.397707230493));
#70653=CARTESIAN_POINT('Ctrl Pts',(-17.2559605706217,-20.4676446069254,
-15.39266782742));
#70654=CARTESIAN_POINT('Ctrl Pts',(-17.2491787063536,-20.4610012748967,
-15.3921019399614));
#70655=CARTESIAN_POINT('Ctrl Pts',(-17.2391915853088,-20.4510856485608,
-15.3912578735231));
#70656=CARTESIAN_POINT('Ctrl Pts',(-17.2359517887871,-20.4478480986818,
-15.3909823647082));
#70657=CARTESIAN_POINT('Ctrl Pts',(-17.230204245092,-20.4420671412002,-15.3904905149705));
#70658=CARTESIAN_POINT('Ctrl Pts',(-17.2276924031895,-20.439527875814,-15.3902745028146));
#70659=CARTESIAN_POINT('Ctrl Pts',(-17.2223035852484,-20.4340525788117,
-15.3898087770304));
#70660=CARTESIAN_POINT('Ctrl Pts',(-17.2194287728867,-20.4311145642146,
-15.3895589076406));
#70661=CARTESIAN_POINT('Ctrl Pts',(-17.2115116896153,-20.4229761431723,
-15.3888669086129));
#70662=CARTESIAN_POINT('Ctrl Pts',(-17.2064875802117,-20.4177582586973,
-15.3884234064824));
#70663=CARTESIAN_POINT('Ctrl Pts',(-17.1790231774189,-20.3889400224135,
-15.3859754000312));
#70664=CARTESIAN_POINT('Ctrl Pts',(-17.1571042851005,-20.3648514363793,
-15.3839344879802));
#70665=CARTESIAN_POINT('Ctrl Pts',(-17.0290710793708,-20.2174527716086,
-15.3715278443063));
#70666=CARTESIAN_POINT('Ctrl Pts',(-16.9369053699052,-20.0827538043303,
-15.3605726816256));
#70667=CARTESIAN_POINT('Ctrl Pts',(-16.8066268175575,-19.8354954811239,
-15.342317278926));
#70668=CARTESIAN_POINT('Ctrl Pts',(-16.7608186066422,-19.7278186919677,
-15.334877095808));
#70669=CARTESIAN_POINT('Ctrl Pts',(-16.7196357931291,-19.6033294279771,
-15.3268706501961));
#70670=CARTESIAN_POINT('Ctrl Pts',(-16.7152852994567,-19.5897179276128,
-15.3260026821719));
#70671=CARTESIAN_POINT('Ctrl Pts',(-16.7085806030627,-19.5679843704653,
-15.324628383856));
#70672=CARTESIAN_POINT('Ctrl Pts',(-16.7061367273819,-19.559890638975,-15.3241191255642));
#70673=CARTESIAN_POINT('Ctrl Pts',(-16.7019120782303,-19.5455902352014,
-15.3232237501348));
#70674=CARTESIAN_POINT('Ctrl Pts',(-16.7001111036489,-19.5393896899517,
-15.3228369768826));
#70675=CARTESIAN_POINT('Ctrl Pts',(-16.6964447782729,-19.5265479108118,
-15.3220389076684));
#70676=CARTESIAN_POINT('Ctrl Pts',(-16.6945834615177,-19.5199055975265,
-15.3216277470936));
#70677=CARTESIAN_POINT('Ctrl Pts',(-16.6898890436285,-19.5028323033913,
-15.3205750324749));
#70678=CARTESIAN_POINT('Ctrl Pts',(-16.687103279785,-19.4923884267351,-15.3199350197606));
#70679=CARTESIAN_POINT('Ctrl Pts',(-16.6758102403467,-19.4487099715188,
-15.3172743162655));
#70680=CARTESIAN_POINT('Ctrl Pts',(-16.6680311637819,-19.4152913197268,
-15.3152771550845));
#70681=CARTESIAN_POINT('Ctrl Pts',(-16.6498822265504,-19.327737688799,-15.3101329729858));
#70682=CARTESIAN_POINT('Ctrl Pts',(-16.640807658563,-19.2733598786047,-15.3070253431617));
#70683=CARTESIAN_POINT('Ctrl Pts',(-16.6200900354575,-19.1102104048834,
-15.2978808090869));
#70684=CARTESIAN_POINT('Ctrl Pts',(-16.6147400597023,-19.0008268301613,
-15.2919926338135));
#70685=CARTESIAN_POINT('Ctrl Pts',(-16.6191736214412,-18.8457009827542,
-15.2835434786426));
#70686=CARTESIAN_POINT('Ctrl Pts',(-16.6219708881489,-18.7999378945219,
-15.2810371418153));
#70687=CARTESIAN_POINT('Ctrl Pts',(-16.6283556988882,-18.7318661195058,
-15.2772456994723));
#70688=CARTESIAN_POINT('Ctrl Pts',(-16.6308182625417,-18.7094646886026,
-15.2759876589647));
#70689=CARTESIAN_POINT('Ctrl Pts',(-16.6343888314768,-18.6811532594336,
-15.2743800372108));
#70690=CARTESIAN_POINT('Ctrl Pts',(-16.6351650644398,-18.6752023699536,
-15.2740411320029));
#70691=CARTESIAN_POINT('Ctrl Pts',(-16.6420724354838,-18.6239480927944,
-15.2711130222594));
#70692=CARTESIAN_POINT('Ctrl Pts',(-16.6496438015094,-18.578854508832,-15.2684752227161));
#70693=CARTESIAN_POINT('Ctrl Pts',(-16.6601732546215,-18.5265710909261,
-15.2653079566838));
#70694=CARTESIAN_POINT('Ctrl Pts',(-16.6617187981786,-18.5191053902604,
-15.2648530790375));
#70695=CARTESIAN_POINT('Ctrl Pts',(-16.66426314209,-18.5071409501252,-15.2641196620535));
#70696=CARTESIAN_POINT('Ctrl Pts',(-16.6652363801142,-18.5026367623359,
-15.2638425453159));
#70697=CARTESIAN_POINT('Ctrl Pts',(-16.6669925174339,-18.494635914592,-15.2633484426436));
#70698=CARTESIAN_POINT('Ctrl Pts',(-16.6677695966785,-18.4911380251998,
-15.2631317922469));
#70699=CARTESIAN_POINT('Ctrl Pts',(-16.6694428448938,-18.4836954878489,
-15.2626694507465));
#70700=CARTESIAN_POINT('Ctrl Pts',(-16.6703414263075,-18.4797514919101,
-15.2624236285701));
#70701=CARTESIAN_POINT('Ctrl Pts',(-16.6728139530036,-18.4690410555934,
-15.2617538953122));
#70702=CARTESIAN_POINT('Ctrl Pts',(-16.6744098945089,-18.4622798180716,
-15.2613287509825));
#70703=CARTESIAN_POINT('Ctrl Pts',(-16.6827294761852,-18.4277938285908,
-15.2591486617646));
#70704=CARTESIAN_POINT('Ctrl Pts',(-16.6899794236814,-18.4002006072036,
-15.2573659075871));
#70705=CARTESIAN_POINT('Ctrl Pts',(-16.7129483545565,-18.3194568455118,
-15.2520523826054));
#70706=CARTESIAN_POINT('Ctrl Pts',(-16.730198957188,-18.2667692837795,-15.2484607159687));
#70707=CARTESIAN_POINT('Ctrl Pts',(-16.7980417738446,-18.0841341650226,
-15.2356998065876));
#70708=CARTESIAN_POINT('Ctrl Pts',(-16.8593845123562,-17.9585478960011,
-15.2263847169485));
#70709=CARTESIAN_POINT('Ctrl Pts',(-16.9799883621592,-17.7631941414895,
-15.2115627947521));
#70710=CARTESIAN_POINT('Ctrl Pts',(-17.0322022829082,-17.6895799289483,
-15.2058809790918));
#70711=CARTESIAN_POINT('Ctrl Pts',(-17.0975939666049,-17.6088497740306,
-15.199542103372));
#70712=CARTESIAN_POINT('Ctrl Pts',(-17.1063331811176,-17.5982725620446,
-15.1987091711963));
#70713=CARTESIAN_POINT('Ctrl Pts',(-17.1205158216737,-17.5814429958551,
-15.1973797690614));
#70714=CARTESIAN_POINT('Ctrl Pts',(-17.1258941064206,-17.575136487009,-15.1968806613508));
#70715=CARTESIAN_POINT('Ctrl Pts',(-17.1355107893663,-17.5639933010039,
-15.1959970247908));
#70716=CARTESIAN_POINT('Ctrl Pts',(-17.1397344247621,-17.5591440742142,
-15.1956118940241));
#70717=CARTESIAN_POINT('Ctrl Pts',(-17.1485820545855,-17.5490789318872,
-15.1948112263512));
#70718=CARTESIAN_POINT('Ctrl Pts',(-17.1532098515782,-17.5438664504261,
-15.1943958545485));
#70719=CARTESIAN_POINT('Ctrl Pts',(-17.1652981621679,-17.5303855776059,
-15.1933196288962));
#70720=CARTESIAN_POINT('Ctrl Pts',(-17.1727983867463,-17.522152962056,-15.1926604536255));
#70721=CARTESIAN_POINT('Ctrl Pts',(-17.2056823888846,-17.4866250945433,
-15.1898067800555));
#70722=CARTESIAN_POINT('Ctrl Pts',(-17.2317205046333,-17.4599427283636,
-15.1876403909399));
#70723=CARTESIAN_POINT('Ctrl Pts',(-17.3027982590784,-17.3908544570607,
-15.1819520632266));
#70724=CARTESIAN_POINT('Ctrl Pts',(-17.349015341122,-17.3497103305656,-15.1784813768306));
#70725=CARTESIAN_POINT('Ctrl Pts',(-17.5080711926025,-17.2201450973463,
-15.1671327179264));
#70726=CARTESIAN_POINT('Ctrl Pts',(-17.6280672587318,-17.1411623411707,
-15.1595222932053));
#70727=CARTESIAN_POINT('Ctrl Pts',(-17.8209694150088,-17.0405659631828,
-15.1474692355978));
#70728=CARTESIAN_POINT('Ctrl Pts',(-17.8885766653055,-17.0097173607798,
-15.1432689572719));
#70729=CARTESIAN_POINT('Ctrl Pts',(-17.9664518545203,-16.9790204699717,
-15.1383075629105));
#70730=CARTESIAN_POINT('Ctrl Pts',(-17.9752703218368,-16.9756124748641,
-15.1377439976544));
#70731=CARTESIAN_POINT('Ctrl Pts',(-17.9883871164501,-16.9706440664972,
-15.1369027392614));
#70732=CARTESIAN_POINT('Ctrl Pts',(-17.9926682888784,-16.9690382755767,
-15.1366276905548));
#70733=CARTESIAN_POINT('Ctrl Pts',(-18.0003022405588,-16.9662030943809,
-15.1361363434057));
#70734=CARTESIAN_POINT('Ctrl Pts',(-18.0036529607038,-16.9649683056048,
-15.1359203711214));
#70735=CARTESIAN_POINT('Ctrl Pts',(-18.0108722935925,-16.9623286051126,
-15.1354543665416));
#70736=CARTESIAN_POINT('Ctrl Pts',(-18.0147418274363,-16.9609265156853,
-15.1352041765559));
#70737=CARTESIAN_POINT('Ctrl Pts',(-18.0254550431428,-16.9570799876455,
-15.134510406041));
#70738=CARTESIAN_POINT('Ctrl Pts',(-18.0323071852899,-16.9546595177993,
-15.1340654416635));
#70739=CARTESIAN_POINT('Ctrl Pts',(-18.070262434483,-16.9414715145958,-15.1315944476733));
#70740=CARTESIAN_POINT('Ctrl Pts',(-18.1015991007315,-16.9313958400787,
-15.1295312164146));
#70741=CARTESIAN_POINT('Ctrl Pts',(-18.2888648410165,-16.8759669699032,
-15.1171169597771));
#70742=CARTESIAN_POINT('Ctrl Pts',(-18.4493551482041,-16.8479477810541,
-15.1061821037736));
#70743=CARTESIAN_POINT('Ctrl Pts',(-18.7279782325901,-16.8317942015676,
-15.087952777577));
#70744=CARTESIAN_POINT('Ctrl Pts',(-18.8448602567619,-16.8346840862477,
-15.080519090292));
#70745=CARTESIAN_POINT('Ctrl Pts',(-18.975130882362,-16.8487289660873,-15.0725186922775));
#70746=CARTESIAN_POINT('Ctrl Pts',(-18.9893208711825,-16.850404317435,-15.0716508042757));
#70747=CARTESIAN_POINT('Ctrl Pts',(-19.0118784083963,-16.8532994349065,
-15.0702766083134));
#70748=CARTESIAN_POINT('Ctrl Pts',(-19.0202572980912,-16.8544258691753,
-15.0697673730315));
#70749=CARTESIAN_POINT('Ctrl Pts',(-19.0350231259204,-16.8565010699138,
-15.068872024366));
#70750=CARTESIAN_POINT('Ctrl Pts',(-19.0414128501888,-16.8574289151946,
-15.0684852549911));
#70751=CARTESIAN_POINT('Ctrl Pts',(-19.0546203077015,-16.8594084957146,
-15.0676871806656));
#70752=CARTESIAN_POINT('Ctrl Pts',(-19.0614373529596,-16.8604643519326,
-15.0672760111667));
#70753=CARTESIAN_POINT('Ctrl Pts',(-19.0789230127468,-16.8632601984035,
-15.0662232465561));
#70754=CARTESIAN_POINT('Ctrl Pts',(-19.0895837652939,-16.8650486263655,
-15.0655831930613));
#70755=CARTESIAN_POINT('Ctrl Pts',(-19.1340249684607,-16.8728544245807,
-15.0629220931672));
#70756=CARTESIAN_POINT('Ctrl Pts',(-19.167671425178,-16.8796111390781,-15.0609245853173));
#70757=CARTESIAN_POINT('Ctrl Pts',(-19.2549012942788,-16.8993458582374,
-15.055779308439));
#70758=CARTESIAN_POINT('Ctrl Pts',(-19.3081692601104,-16.9136041869511,
-15.052670952495));
#70759=CARTESIAN_POINT('Ctrl Pts',(-19.4636262519155,-16.9617943301914,
-15.0436213041689));
#70760=CARTESIAN_POINT('Ctrl Pts',(-19.5638523666862,-17.0014567341608,
-15.0378222665605));
#70761=CARTESIAN_POINT('Ctrl Pts',(-19.7686997248433,-17.1011804358314,
-15.025422299592));
#70762=CARTESIAN_POINT('Ctrl Pts',(-19.8720797850926,-17.1628933623888,
-15.0188266624207));
#70763=CARTESIAN_POINT('Ctrl Pts',(-19.977364919844,-17.2385756668261,-15.0111420220576));
#70764=CARTESIAN_POINT('Ctrl Pts',(-19.9850420139582,-17.2441729768176,
-15.0105757005653));
#70765=CARTESIAN_POINT('Ctrl Pts',(-19.9963649030556,-17.2525457219582,
-15.009731109385));
#70766=CARTESIAN_POINT('Ctrl Pts',(-20.0000399049371,-17.2552817117086,
-15.0094555146848));
#70767=CARTESIAN_POINT('Ctrl Pts',(-20.0064390939317,-17.2600781876615,
-15.0089729992529));
#70768=CARTESIAN_POINT('Ctrl Pts',(-20.0091672108293,-17.2621333629289,
-15.0087664512564));
#70769=CARTESIAN_POINT('Ctrl Pts',(-20.0150561291599,-17.2665920490921,
-15.0083187585703));
#70770=CARTESIAN_POINT('Ctrl Pts',(-20.0182150982555,-17.268997817038,-15.0080774586215));
#70771=CARTESIAN_POINT('Ctrl Pts',(-20.0266048131899,-17.2754245242627,
-15.0074335907187));
#70772=CARTESIAN_POINT('Ctrl Pts',(-20.0318235126544,-17.2794610150206,
-15.0070299489986));
#70773=CARTESIAN_POINT('Ctrl Pts',(-20.0434206209078,-17.2885179512195,
-15.0061261168653));
#70774=CARTESIAN_POINT('Ctrl Pts',(-20.0497891623606,-17.2935507952878,
-15.0056251116606));
#70775=CARTESIAN_POINT('Ctrl Pts',(-20.0690118635665,-17.3089222656419,
-15.0040990779448));
#70776=CARTESIAN_POINT('Ctrl Pts',(-20.0817739702814,-17.3193743826084,
-15.003067040158));
#70777=CARTESIAN_POINT('Ctrl Pts',(-20.1289504563412,-17.358941859414,-14.9991849236106));
#70778=CARTESIAN_POINT('Ctrl Pts',(-20.1625525541588,-17.389003488229,-14.9962845061265));
#70779=CARTESIAN_POINT('Ctrl Pts',(-20.2500826201925,-17.4724926968091,
-14.9884117506999));
#70780=CARTESIAN_POINT('Ctrl Pts',(-20.3021401358658,-17.5277864305359,
-14.9833857751019));
#70781=CARTESIAN_POINT('Ctrl Pts',(-20.4510375815278,-17.7040243071374,
-14.9681454430927));
#70782=CARTESIAN_POINT('Ctrl Pts',(-20.5377009563585,-17.832919720385,-14.9580580753843));
#70783=CARTESIAN_POINT('Ctrl Pts',(-20.6206412514692,-17.9913506668948,
-14.947040598894));
#70784=CARTESIAN_POINT('Ctrl Pts',(-20.6313864541042,-18.012751858876,-14.9455779571933));
#70785=CARTESIAN_POINT('Ctrl Pts',(-20.645973430585,-18.0430771293405,-14.94354034568));
#70786=CARTESIAN_POINT('Ctrl Pts',(-20.6501201139051,-18.0518517355091,
-14.9429548089173));
#70787=CARTESIAN_POINT('Ctrl Pts',(-20.6567308726811,-18.0660931530048,
-14.9420109045188));
#70788=CARTESIAN_POINT('Ctrl Pts',(-20.6592322829528,-18.0715423870848,
-14.9416512493241));
#70789=CARTESIAN_POINT('Ctrl Pts',(-20.664397467424,-18.0829218222117,-14.9409033130694));
#70790=CARTESIAN_POINT('Ctrl Pts',(-20.6670571477576,-18.0888538210115,
-14.9405151759685));
#70791=CARTESIAN_POINT('Ctrl Pts',(-20.6732798987867,-18.1029057179177,
-14.9395998383254));
#70792=CARTESIAN_POINT('Ctrl Pts',(-20.6768193795688,-18.1110359771549,
-14.9390734498376));
#70793=CARTESIAN_POINT('Ctrl Pts',(-20.6883951620446,-18.1380889539118,
-14.937332370114));
#70794=CARTESIAN_POINT('Ctrl Pts',(-20.6962070636656,-18.1571068476923,
-14.9361253045819));
#70795=CARTESIAN_POINT('Ctrl Pts',(-20.736185600108,-18.2586162775481,-14.9297670310457));
#70796=CARTESIAN_POINT('Ctrl Pts',(-20.7634324080283,-18.3429557947427,
-14.9247830122503));
#70797=CARTESIAN_POINT('Ctrl Pts',(-20.8290276887774,-18.6001176753881,
-14.9101344054699));
#70798=CARTESIAN_POINT('Ctrl Pts',(-20.851085988477,-18.7762442174503,-14.9008595449284));
#70799=CARTESIAN_POINT('Ctrl Pts',(-20.850999748114,-18.9530327076519,-14.890777192852));
#70800=CARTESIAN_POINT('Ctrl Pts',(-20.8509997467307,-18.9530355395134,
-14.8907770313492));
#70801=CARTESIAN_POINT('Ctrl Pts',(-20.8509866388438,-18.9798325789464,
-14.889248779021));
#70802=CARTESIAN_POINT('Ctrl Pts',(-20.8504647357704,-19.0066259838651,
-14.8877018299672));
#70803=CARTESIAN_POINT('Ctrl Pts',(-20.8488772347909,-19.0478815498525,
-14.8852810116848));
#70804=CARTESIAN_POINT('Ctrl Pts',(-20.8481713904245,-19.0623553181648,
-14.8844243242303));
#70805=CARTESIAN_POINT('Ctrl Pts',(-20.8470399810294,-19.081511077281,-14.883279390487));
#70806=CARTESIAN_POINT('Ctrl Pts',(-20.8467473096707,-19.086200913193,-14.8829981965203));
#70807=CARTESIAN_POINT('Ctrl Pts',(-20.8462061821127,-19.0944311785953,
-14.8825031124846));
#70808=CARTESIAN_POINT('Ctrl Pts',(-20.845964430651,-19.0979720508692,-14.8822895904033));
#70809=CARTESIAN_POINT('Ctrl Pts',(-20.845471825666,-19.1049296118924,-14.8818689752654));
#70810=CARTESIAN_POINT('Ctrl Pts',(-20.8452215797263,-19.1083463397607,
-14.881661915791));
#70811=CARTESIAN_POINT('Ctrl Pts',(-20.844666932587,-19.1156749680097,-14.8812166858999));
#70812=CARTESIAN_POINT('Ctrl Pts',(-20.8443599504657,-19.1195866174848,
-14.8809783745506));
#70813=CARTESIAN_POINT('Ctrl Pts',(-20.8435234725452,-19.1298783426118,
-14.8803496430295));
#70814=CARTESIAN_POINT('Ctrl Pts',(-20.8429759117084,-19.1362568516816,
-14.8799582295632));
#70815=CARTESIAN_POINT('Ctrl Pts',(-20.8405832034925,-19.1627202290814,
-14.8783273541142));
#70816=CARTESIAN_POINT('Ctrl Pts',(-20.8384800664517,-19.1827799588661,
-14.8770744599677));
#70817=CARTESIAN_POINT('Ctrl Pts',(-20.8355857381717,-19.2070383408862,
-14.8755415821871));
#70818=CARTESIAN_POINT('Ctrl Pts',(-20.835067953567,-19.2112694045152,-14.8752735671886));
#70819=CARTESIAN_POINT('Ctrl Pts',(-20.8313092268496,-19.2412328988615,
-14.873371027654));
#70820=CARTESIAN_POINT('Ctrl Pts',(-20.8276085505026,-19.2669044098143,
-14.8717174315256));
#70821=CARTESIAN_POINT('Ctrl Pts',(-20.8020054287801,-19.4240147384879,
-14.8614773343571));
#70822=CARTESIAN_POINT('Ctrl Pts',(-20.7682211192295,-19.5531157516609,
-14.8525677751688));
#70823=CARTESIAN_POINT('Ctrl Pts',(-20.7225805876025,-19.6781103542923,
-14.843838552956));
#70824=CARTESIAN_POINT('Origin',(-18.734,-18.952,0.));
#70825=CARTESIAN_POINT('',(-20.7225805863163,-19.6781103578147,-14.0426552896606));
#70826=CARTESIAN_POINT('',(-20.7225805821191,-19.6781103693095,-14.2664527148047));
#70827=CARTESIAN_POINT('',(-20.7225805821191,-19.6781103693095,0.));
#70828=CARTESIAN_POINT('',(-20.8484261850221,-18.9515327934241,-14.3109440134296));
#70829=CARTESIAN_POINT('Ctrl Pts',(-20.7225805821191,-19.6781103693095,
-14.2664527148047));
#70830=CARTESIAN_POINT('Ctrl Pts',(-20.7483493346654,-19.607538121474,-14.2709758300142));
#70831=CARTESIAN_POINT('Ctrl Pts',(-20.7703906773062,-19.5355010802264,
-14.2754989452236));
#70832=CARTESIAN_POINT('Ctrl Pts',(-20.788547932122,-19.4624133566172,-14.2800220604331));
#70833=CARTESIAN_POINT('Ctrl Pts',(-20.806681898482,-19.3894193751646,-14.2845393743048));
#70834=CARTESIAN_POINT('Ctrl Pts',(-20.8209415735944,-19.3153778114031,
-14.2890566881764));
#70835=CARTESIAN_POINT('Ctrl Pts',(-20.8312196579543,-19.2407190785,-14.2935740020481));
#70836=CARTESIAN_POINT('Ctrl Pts',(-20.8414842436756,-19.166158398038,-14.2980853831422));
#70837=CARTESIAN_POINT('Ctrl Pts',(-20.847777586069,-19.0909825928347,-14.3025967642363));
#70838=CARTESIAN_POINT('Ctrl Pts',(-20.8500434700713,-19.0156320105649,
-14.3071081453305));
#70839=CARTESIAN_POINT('Ctrl Pts',(-20.850685621504,-18.994277658663,-14.3083866705462));
#70840=CARTESIAN_POINT('Ctrl Pts',(-20.851004622492,-18.9729093192271,-14.3096651957618));
#70841=CARTESIAN_POINT('Ctrl Pts',(-20.850999949394,-18.9515371115436,-14.3109437209775));
#70842=CARTESIAN_POINT('Ctrl Pts',(-20.8476070208165,-18.9515314190757,
-14.3109441065097));
#70843=CARTESIAN_POINT('Ctrl Pts',(-20.8482398705352,-18.6260442197703,
-14.3304466040445));
#70844=CARTESIAN_POINT('Ctrl Pts',(-20.6243346302329,-17.5938833017488,
-14.3923410371397));
#70845=CARTESIAN_POINT('Ctrl Pts',(-19.0148744663066,-16.4645435790994,
-14.4966274057954));
#70846=CARTESIAN_POINT('Ctrl Pts',(-16.7944748199427,-17.3694160408942,
-14.6238032124768));
#70847=CARTESIAN_POINT('Ctrl Pts',(-16.3534691457724,-19.7262110589277,
-14.7509790191583));
#70848=CARTESIAN_POINT('Ctrl Pts',(-18.0964527779473,-21.3727154833541,
-14.8781548258396));
#70849=CARTESIAN_POINT('Ctrl Pts',(-20.0208838098492,-20.8979083957969,
-14.9832889543559));
#70850=CARTESIAN_POINT('Ctrl Pts',(-20.6031709075902,-19.9961147240441,
-15.0460311473117));
#70851=CARTESIAN_POINT('Ctrl Pts',(-20.7193262595591,-19.6769292106295,
-15.0663814047069));
#70852=CARTESIAN_POINT('Ctrl Pts',(-20.7225805876025,-19.6781103542923,
-14.843838552956));
#70853=CARTESIAN_POINT('Ctrl Pts',(-20.7076429479187,-19.7190197010936,
-14.8409815753642));
#70854=CARTESIAN_POINT('Ctrl Pts',(-20.6914352889252,-19.7594890121212,
-14.8381415685881));
#70855=CARTESIAN_POINT('Ctrl Pts',(-20.6503533962779,-19.8535323811849,
-14.8315248819409));
#70856=CARTESIAN_POINT('Ctrl Pts',(-20.624479739026,-19.9065985147269,-14.8277783969357));
#70857=CARTESIAN_POINT('Ctrl Pts',(-20.5792836655683,-19.9902275033178,
-14.8218610376395));
#70858=CARTESIAN_POINT('Ctrl Pts',(-20.5613390236455,-20.0214954410477,
-14.8196452307213));
#70859=CARTESIAN_POINT('Ctrl Pts',(-20.5368846514892,-20.0616923074862,
-14.8167904057333));
#70860=CARTESIAN_POINT('Ctrl Pts',(-20.5310922292495,-20.071048529154,-14.8161254489431));
#70861=CARTESIAN_POINT('Ctrl Pts',(-20.5215274852216,-20.0862321927493,
-14.8150454412858));
#70862=CARTESIAN_POINT('Ctrl Pts',(-20.5177990428995,-20.092086906261,-14.8146287798552));
#70863=CARTESIAN_POINT('Ctrl Pts',(-20.5105556221584,-20.1033386128491,
-14.8138275671119));
#70864=CARTESIAN_POINT('Ctrl Pts',(-20.5070446818932,-20.1087381023746,
-14.8134428716056));
#70865=CARTESIAN_POINT('Ctrl Pts',(-20.4989237545119,-20.1211034658168,
-14.8125613564739));
#70866=CARTESIAN_POINT('Ctrl Pts',(-20.4942970518485,-20.128058274632,-14.8120651696503));
#70867=CARTESIAN_POINT('Ctrl Pts',(-20.4818391206991,-20.1465466725458,
-14.8107449666183));
#70868=CARTESIAN_POINT('Ctrl Pts',(-20.4739348442708,-20.1580307194631,
-14.8099237119911));
#70869=CARTESIAN_POINT('Ctrl Pts',(-20.4094818015417,-20.2497212487156,
-14.8033548184419));
#70870=CARTESIAN_POINT('Ctrl Pts',(-20.3475282622321,-20.3259904575298,
-14.7978251132188));
#70871=CARTESIAN_POINT('Ctrl Pts',(-20.1871027224722,-20.4976021845072,
-14.7848692884694));
#70872=CARTESIAN_POINT('Ctrl Pts',(-20.0842495616095,-20.5882204381158,
-14.7775931152199));
#70873=CARTESIAN_POINT('Ctrl Pts',(-19.9317575763164,-20.6983394739842,
-14.7671707328954));
#70874=CARTESIAN_POINT('Ctrl Pts',(-19.8890588089683,-20.7268699132003,
-14.76428429342));
#70875=CARTESIAN_POINT('Ctrl Pts',(-19.8300417414095,-20.7632718679851,
-14.760278081994));
#70876=CARTESIAN_POINT('Ctrl Pts',(-19.8145955360426,-20.7725291874119,
-14.7592280529012));
#70877=CARTESIAN_POINT('Ctrl Pts',(-19.7915638375836,-20.7859363225787,
-14.7576572942295));
#70878=CARTESIAN_POINT('Ctrl Pts',(-19.7840676019868,-20.7902387580534,
-14.7571452683562));
#70879=CARTESIAN_POINT('Ctrl Pts',(-19.7704475716356,-20.7979454269309,
-14.7562131580613));
#70880=CARTESIAN_POINT('Ctrl Pts',(-19.7643327808252,-20.801365416998,-14.7557940299349));
#70881=CARTESIAN_POINT('Ctrl Pts',(-19.7546715390116,-20.8067061425825,
-14.7551306118184));
#70882=CARTESIAN_POINT('Ctrl Pts',(-19.7511363194201,-20.8086472397777,
-14.7548876027571));
#70883=CARTESIAN_POINT('Ctrl Pts',(-19.7475865136736,-20.8105831645117,
-14.7546433163214));
#70884=CARTESIAN_POINT('Ctrl Pts',(-19.747577419482,-20.8105881240403,-14.754642690486));
#70885=CARTESIAN_POINT('Ctrl Pts',(-19.7475591760445,-20.8105980729476,
-14.7546414350229));
#70886=CARTESIAN_POINT('Ctrl Pts',(-19.7475500259468,-20.8106030627899,
-14.7546408053366));
#70887=CARTESIAN_POINT('Ctrl Pts',(-19.7475316696383,-20.8106130728987,
-14.7546395420987));
#70888=CARTESIAN_POINT('Ctrl Pts',(-19.7475224644028,-20.8106180926325,
-14.7546389086143));
#70889=CARTESIAN_POINT('Ctrl Pts',(-19.7475039978208,-20.81062816252,-14.7546376377802));
#70890=CARTESIAN_POINT('Ctrl Pts',(-19.7474947359349,-20.8106332129669,
-14.7546370003935));
#70891=CARTESIAN_POINT('Ctrl Pts',(-19.7474761561388,-20.8106433442301,
-14.7546357217607));
#70892=CARTESIAN_POINT('Ctrl Pts',(-19.7474668377156,-20.8106484253251,
-14.7546350804794));
#70893=CARTESIAN_POINT('Ctrl Pts',(-19.7474481437399,-20.8106586184838,
-14.7546337939814));
#70894=CARTESIAN_POINT('Ctrl Pts',(-19.7474387687128,-20.81066373026,-14.7546331488008));
#70895=CARTESIAN_POINT('Ctrl Pts',(-19.7474199615284,-20.8106739847782,
-14.7546318545042));
#70896=CARTESIAN_POINT('Ctrl Pts',(-19.7474105287671,-20.8106791278484,
-14.7546312053465));
#70897=CARTESIAN_POINT('Ctrl Pts',(-19.7473916056544,-20.8106894452022,
-14.754629903064));
#70898=CARTESIAN_POINT('Ctrl Pts',(-19.7473821153389,-20.810694619465,-14.7546292499416));
#70899=CARTESIAN_POINT('Ctrl Pts',(-19.7473630763891,-20.8107049995977,
-14.7546279396793));
#70900=CARTESIAN_POINT('Ctrl Pts',(-19.7473535279432,-20.8107102053638,
-14.7546272825524));
#70901=CARTESIAN_POINT('Ctrl Pts',(-19.7473343726346,-20.8107206485529,
-14.7546259642743));
#70902=CARTESIAN_POINT('Ctrl Pts',(-19.7473247654062,-20.8107258861743,
-14.7546253030979));
#70903=CARTESIAN_POINT('Ctrl Pts',(-19.7473054912954,-20.8107363937449,
-14.7546239766356));
#70904=CARTESIAN_POINT('Ctrl Pts',(-19.7472958255505,-20.8107416630729,
-14.7546233114281));
#70905=CARTESIAN_POINT('Ctrl Pts',(-19.7472764350954,-20.810752233678,-14.7546219769507));
#70906=CARTESIAN_POINT('Ctrl Pts',(-19.7472667091036,-20.8107575356526,
-14.7546213075927));
#70907=CARTESIAN_POINT('Ctrl Pts',(-19.7472472344797,-20.8107681517453,
-14.7546199673145));
#70908=CARTESIAN_POINT('Ctrl Pts',(-19.7472374305908,-20.8107734959849,
-14.7546192925911));
#70909=CARTESIAN_POINT('Ctrl Pts',(-19.7472177802483,-20.8107842074636,
-14.7546179402112));
#70910=CARTESIAN_POINT('Ctrl Pts',(-19.7472079349286,-20.8107895740844,
-14.7546172626324));
#70911=CARTESIAN_POINT('Ctrl Pts',(-19.7471881820861,-20.8108003410291,
-14.7546159031897));
#70912=CARTESIAN_POINT('Ctrl Pts',(-19.7471782761647,-20.8108057404787,
-14.7546152214359));
#70913=CARTESIAN_POINT('Ctrl Pts',(-19.7471583681398,-20.8108165915978,
-14.7546138513045));
#70914=CARTESIAN_POINT('Ctrl Pts',(-19.7471484177377,-20.8108220150849,
-14.7546131664853));
#70915=CARTESIAN_POINT('Ctrl Pts',(-19.7441389748456,-20.8124622869553,
-14.7544060460706));
#70916=CARTESIAN_POINT('Ctrl Pts',(-19.7411355938517,-20.8140898379721,
-14.7541991424452));
#70917=CARTESIAN_POINT('Ctrl Pts',(-19.7340941498551,-20.8178836217641,
-14.753713597222));
#70918=CARTESIAN_POINT('Ctrl Pts',(-19.7300529967498,-20.820044010535,-14.7534345892217));
#70919=CARTESIAN_POINT('Ctrl Pts',(-19.717608152335,-20.8266451251454,-14.7525743807906));
#70920=CARTESIAN_POINT('Ctrl Pts',(-19.7091816775884,-20.8310423173854,
-14.7519905381892));
#70921=CARTESIAN_POINT('Ctrl Pts',(-19.5939549276201,-20.890187340136,-14.7439909203515));
#70922=CARTESIAN_POINT('Ctrl Pts',(-19.4827287343374,-20.9358072622843,
-14.736094938836));
#70923=CARTESIAN_POINT('Ctrl Pts',(-19.2644117655886,-21.0043641695455,
-14.7209775300448));
#70924=CARTESIAN_POINT('Ctrl Pts',(-19.1582022660974,-21.0289186894102,
-14.7137839202715));
#70925=CARTESIAN_POINT('Ctrl Pts',(-18.9765737644231,-21.0563876931189,
-14.7019827741361));
#70926=CARTESIAN_POINT('Ctrl Pts',(-18.9020306614998,-21.0636480343663,
-14.6972748127376));
#70927=CARTESIAN_POINT('Ctrl Pts',(-18.8084892403596,-21.0677724540655,
-14.6915390227631));
#70928=CARTESIAN_POINT('Ctrl Pts',(-18.7897158813092,-21.0683500420688,
-14.6903963324862));
#70929=CARTESIAN_POINT('Ctrl Pts',(-18.7623887108473,-21.0688269116208,
-14.6887448553477));
#70930=CARTESIAN_POINT('Ctrl Pts',(-18.7538396662056,-21.0689242980466,
-14.6882298932722));
#70931=CARTESIAN_POINT('Ctrl Pts',(-18.7388418088678,-21.0690042842168,
-14.6873293712608));
#70932=CARTESIAN_POINT('Ctrl Pts',(-18.7323932727385,-21.0690092116853,
-14.6869431170728));
#70933=CARTESIAN_POINT('Ctrl Pts',(-18.7198657866567,-21.0689615439237,
-14.6861945317473));
#70934=CARTESIAN_POINT('Ctrl Pts',(-18.7137868941591,-21.0689122291623,
-14.6858321017005));
#70935=CARTESIAN_POINT('Ctrl Pts',(-18.6992460283344,-21.0687316272221,
-14.6849670727568));
#70936=CARTESIAN_POINT('Ctrl Pts',(-18.6907844222653,-21.0685757811215,
-14.684465246086));
#70937=CARTESIAN_POINT('Ctrl Pts',(-18.6601984170295,-21.0678289520878,
-14.682656722482));
#70938=CARTESIAN_POINT('Ctrl Pts',(-18.6380821998677,-21.0669417623734,
-14.6813592826769));
#70939=CARTESIAN_POINT('Ctrl Pts',(-18.4309232207095,-21.0553752570998,
-14.669292435323));
#70940=CARTESIAN_POINT('Ctrl Pts',(-18.2480265114241,-21.0207867967459,
-14.6593770169785));
#70941=CARTESIAN_POINT('Ctrl Pts',(-17.995689099154,-20.937707355755,-14.6448953879912));
#70942=CARTESIAN_POINT('Ctrl Pts',(-17.9209152180251,-20.9082790729295,
-14.6404800235867));
#70943=CARTESIAN_POINT('Ctrl Pts',(-17.8152387635287,-20.8595817102325,
-14.6338245873714));
#70944=CARTESIAN_POINT('Ctrl Pts',(-17.7828712094407,-20.8436510949149,
-14.6317264791834));
#70945=CARTESIAN_POINT('Ctrl Pts',(-17.7443139683167,-20.8234343005845,
-14.6291356243559));
#70946=CARTESIAN_POINT('Ctrl Pts',(-17.7377178184286,-20.8199310998068,
-14.6286891004227));
#70947=CARTESIAN_POINT('Ctrl Pts',(-17.7274769485285,-20.8144225222623,
-14.6279904878432));
#70948=CARTESIAN_POINT('Ctrl Pts',(-17.723819293524,-20.8124411423512,-14.6277398984237));
#70949=CARTESIAN_POINT('Ctrl Pts',(-17.7170371875418,-20.8087413264565,
-14.6272732129449));
#70950=CARTESIAN_POINT('Ctrl Pts',(-17.7139112298574,-20.8070257722518,
-14.6270573006711));
#70951=CARTESIAN_POINT('Ctrl Pts',(-17.7068415732848,-20.803122606612,-14.6265671603556));
#70952=CARTESIAN_POINT('Ctrl Pts',(-17.7029005414877,-20.8009302972441,
-14.6262926350412));
#70953=CARTESIAN_POINT('Ctrl Pts',(-17.6927437972028,-20.7952377511309,
-14.6255818503118));
#70954=CARTESIAN_POINT('Ctrl Pts',(-17.6865387758885,-20.7917186925543,
-14.6251444250928));
#70955=CARTESIAN_POINT('Ctrl Pts',(-17.6485596117781,-20.7699251144456,
-14.6224480069914));
#70956=CARTESIAN_POINT('Ctrl Pts',(-17.6172487745305,-20.75086044076,-14.6201428557126));
#70957=CARTESIAN_POINT('Ctrl Pts',(-17.4431944831213,-20.6385858369582,
-14.6069248159007));
#70958=CARTESIAN_POINT('Ctrl Pts',(-17.3116252437888,-20.5292139370732,
-14.5954219872646));
#70959=CARTESIAN_POINT('Ctrl Pts',(-17.1290835939153,-20.3358495552604,
-14.5781406462631));
#70960=CARTESIAN_POINT('Ctrl Pts',(-17.0683335952191,-20.2620976862588,
-14.5720772490551));
#70961=CARTESIAN_POINT('Ctrl Pts',(-17.0003042799481,-20.1670909392671,
-14.5648995399914));
#70962=CARTESIAN_POINT('Ctrl Pts',(-16.9881112547638,-20.149505483256,-14.5635952934218));
#70963=CARTESIAN_POINT('Ctrl Pts',(-16.9711651700848,-20.1242557553682,
-14.5617562256899));
#70964=CARTESIAN_POINT('Ctrl Pts',(-16.9661915242067,-20.116741769833,-14.5612130911202));
#70965=CARTESIAN_POINT('Ctrl Pts',(-16.957698413396,-20.1037309880657,-14.5602796770699));
#70966=CARTESIAN_POINT('Ctrl Pts',(-16.9541561443926,-20.0982492951273,
-14.5598885463533));
#70967=CARTESIAN_POINT('Ctrl Pts',(-16.9474252612597,-20.0877267621261,
-14.559141777503));
#70968=CARTESIAN_POINT('Ctrl Pts',(-16.9442324952682,-20.0826886642404,
-14.5587859873076));
#70969=CARTESIAN_POINT('Ctrl Pts',(-16.9359919718277,-20.0695629814295,
-14.5578635619645));
#70970=CARTESIAN_POINT('Ctrl Pts',(-16.9309774411911,-20.0614546154661,
-14.5572981579801));
#70971=CARTESIAN_POINT('Ctrl Pts',(-16.9140973996719,-20.0337433043207,
-14.5553805635421));
#70972=CARTESIAN_POINT('Ctrl Pts',(-16.9024951897436,-20.0139812811232,
-14.554037989369));
#70973=CARTESIAN_POINT('Ctrl Pts',(-16.8043356504924,-19.840391151968,-14.5424490358628));
#70974=CARTESIAN_POINT('Ctrl Pts',(-16.7370108230236,-19.6764889356372,
-14.5329638207747));
#70975=CARTESIAN_POINT('Ctrl Pts',(-16.6682205241966,-19.4228393271697,
-14.5186615910465));
#70976=CARTESIAN_POINT('Ctrl Pts',(-16.6507495062445,-19.3382635647562,
-14.5139355675406));
#70977=CARTESIAN_POINT('Ctrl Pts',(-16.6331388704248,-19.2156064655233,
-14.5068593859828));
#70978=CARTESIAN_POINT('Ctrl Pts',(-16.6287843998222,-19.1782139193902,
-14.5046726174139));
#70979=CARTESIAN_POINT('Ctrl Pts',(-16.6247551286356,-19.1331967041538,
-14.5019834456781));
#70980=CARTESIAN_POINT('Ctrl Pts',(-16.6241214149201,-19.1256621008888,
-14.5015314594217));
#70981=CARTESIAN_POINT('Ctrl Pts',(-16.6232000776199,-19.113957278688,-14.500826145076));
#70982=CARTESIAN_POINT('Ctrl Pts',(-16.6228844118202,-19.1097892426324,
-14.5005743630948));
#70983=CARTESIAN_POINT('Ctrl Pts',(-16.6223224748363,-19.1020657577902,
-14.5001066060134));
#70984=CARTESIAN_POINT('Ctrl Pts',(-16.6220728369585,-19.0985106117853,
-14.4998908219755));
#70985=CARTESIAN_POINT('Ctrl Pts',(-16.621529449458,-19.0904820237861,-14.4994024513685));
#70986=CARTESIAN_POINT('Ctrl Pts',(-16.6212409332976,-19.0860082946337,
-14.499129576732));
#70987=CARTESIAN_POINT('Ctrl Pts',(-16.6204331128662,-19.0728306341277,
-14.4983236884368));
#70988=CARTESIAN_POINT('Ctrl Pts',(-16.6199533779791,-19.0641244953032,
-14.4977885384742));
#70989=CARTESIAN_POINT('Ctrl Pts',(-16.6169217648312,-19.0021391715391,
-14.4939602514148));
#70990=CARTESIAN_POINT('Ctrl Pts',(-16.6163308011492,-18.948787721568,-14.4905700676359));
#70991=CARTESIAN_POINT('Ctrl Pts',(-16.6182284094208,-18.8777415637757,
-14.4859767988122));
#70992=CARTESIAN_POINT('Ctrl Pts',(-16.6189249917261,-18.8600140040091,
-14.4848241015923));
#70993=CARTESIAN_POINT('Ctrl Pts',(-16.6223516703974,-18.7939759227892,
-14.480510044686));
#70994=CARTESIAN_POINT('Ctrl Pts',(-16.6265149429976,-18.7457555444233,
-14.4773202259516));
#70995=CARTESIAN_POINT('Ctrl Pts',(-16.6454646084781,-18.5891319441843,
-14.4668986555548));
#70996=CARTESIAN_POINT('Ctrl Pts',(-16.6669999515267,-18.4817154340415,
-14.4596659525143));
#70997=CARTESIAN_POINT('Ctrl Pts',(-16.7117227611718,-18.323414473137,-14.4490925059294));
#70998=CARTESIAN_POINT('Ctrl Pts',(-16.7287683875275,-18.2709919261779,
-14.445603384554));
#70999=CARTESIAN_POINT('Ctrl Pts',(-16.7597139762447,-18.1871075927867,
-14.4400458367904));
#71000=CARTESIAN_POINT('Ctrl Pts',(-16.7723674786205,-18.1552166131295,
-14.4379389720323));
#71001=CARTESIAN_POINT('Ctrl Pts',(-16.7900202330708,-18.113699047025,-14.4352024444129));
#71002=CARTESIAN_POINT('Ctrl Pts',(-16.7943255990543,-18.1037847872798,
-14.434549440251));
#71003=CARTESIAN_POINT('Ctrl Pts',(-16.8015027788911,-18.0875978523182,
-14.4334839409556));
#71004=CARTESIAN_POINT('Ctrl Pts',(-16.8043296188266,-18.0813055620455,
-14.4330699163808));
#71005=CARTESIAN_POINT('Ctrl Pts',(-16.8098619102645,-18.0691504652003,
-14.4322704012817));
#71006=CARTESIAN_POINT('Ctrl Pts',(-16.8125635249759,-18.0632860058831,
-14.4318847844145));
#71007=CARTESIAN_POINT('Ctrl Pts',(-16.8188645674854,-18.0497712285782,
-14.4309963640559));
#71008=CARTESIAN_POINT('Ctrl Pts',(-16.822483094604,-18.0421298969617,-14.4304942266299));
#71009=CARTESIAN_POINT('Ctrl Pts',(-16.8323404074004,-18.021632335304,-14.4291476168919));
#71010=CARTESIAN_POINT('Ctrl Pts',(-16.8386638134609,-18.0088171160672,
-14.4283060859858));
#71011=CARTESIAN_POINT('Ctrl Pts',(-16.8978737344223,-17.8918208441485,
-14.420624308031));
#71012=CARTESIAN_POINT('Ctrl Pts',(-16.9591729457351,-17.7921147917786,
-14.4141007390592));
#71013=CARTESIAN_POINT('Ctrl Pts',(-17.1248209892401,-17.5668178426426,
-14.3987920341743));
#71014=CARTESIAN_POINT('Ctrl Pts',(-17.2360388736691,-17.4472451057684,
-14.3901900912923));
#71015=CARTESIAN_POINT('Ctrl Pts',(-17.3845340351765,-17.3205329979835,
-14.3789809299058));
#71016=CARTESIAN_POINT('Ctrl Pts',(-17.4097099205386,-17.300031933106,-14.3770873619667));
#71017=CARTESIAN_POINT('Ctrl Pts',(-17.4410606641621,-17.2756798507381,
-14.3747237190424));
#71018=CARTESIAN_POINT('Ctrl Pts',(-17.4467983648085,-17.2712700050573,
-14.3742909078512));
#71019=CARTESIAN_POINT('Ctrl Pts',(-17.4558292253301,-17.2644024902162,
-14.3736091340303));
#71020=CARTESIAN_POINT('Ctrl Pts',(-17.4591071853729,-17.2619247961109,
-14.3733615557264));
#71021=CARTESIAN_POINT('Ctrl Pts',(-17.4652481537575,-17.2573110869204,
-14.3728974863215));
#71022=CARTESIAN_POINT('Ctrl Pts',(-17.4681093618142,-17.2551727692675,
-14.3726811603458));
#71023=CARTESIAN_POINT('Ctrl Pts',(-17.4746535600816,-17.250307741221,-14.3721861433191));
#71024=CARTESIAN_POINT('Ctrl Pts',(-17.4783399877556,-17.2475857510388,
-14.3719071300551));
#71025=CARTESIAN_POINT('Ctrl Pts',(-17.4897001517645,-17.2392544735096,
-14.3710468896221));
#71026=CARTESIAN_POINT('Ctrl Pts',(-17.4974027291289,-17.2336849727822,
-14.370463020003));
#71027=CARTESIAN_POINT('Ctrl Pts',(-17.6025137244998,-17.1587551529989,
-14.3624902741026));
#71028=CARTESIAN_POINT('Ctrl Pts',(-17.7055802435141,-17.0977253590708,
-14.3546245546615));
#71029=CARTESIAN_POINT('Ctrl Pts',(-17.9113747828314,-16.9983224336356,
-14.339526361252));
#71030=CARTESIAN_POINT('Ctrl Pts',(-18.0130398286374,-16.9585637235131,
-14.3323218107826));
#71031=CARTESIAN_POINT('Ctrl Pts',(-18.1891373989897,-16.9049412180369,
-14.3204940671805));
#71032=CARTESIAN_POINT('Ctrl Pts',(-18.2620726832091,-16.8869063779302,
-14.3157707365048));
#71033=CARTESIAN_POINT('Ctrl Pts',(-18.3542966735888,-16.8692450197401,
-14.3100183580194));
#71034=CARTESIAN_POINT('Ctrl Pts',(-18.3728205672688,-16.8659529302716,
-14.3088736998168));
#71035=CARTESIAN_POINT('Ctrl Pts',(-18.399828877072,-16.8615235342935,-14.307219920537));
#71036=CARTESIAN_POINT('Ctrl Pts',(-18.408279799198,-16.8601901264174,-14.3067046000093));
#71037=CARTESIAN_POINT('Ctrl Pts',(-18.4231151909209,-16.8579414455019,
-14.3058036645836));
#71038=CARTESIAN_POINT('Ctrl Pts',(-18.4294961488017,-16.8570040572316,
-14.3054173534682));
#71039=CARTESIAN_POINT('Ctrl Pts',(-18.4418980674715,-16.8552400246184,
-14.3046688127312));
#71040=CARTESIAN_POINT('Ctrl Pts',(-18.447918493792,-16.854410119604,-14.304306483472));
#71041=CARTESIAN_POINT('Ctrl Pts',(-18.4623244409392,-16.8524874614138,
-14.3034419416742));
#71042=CARTESIAN_POINT('Ctrl Pts',(-18.4707131409848,-16.8514189989209,
-14.3029404993663));
#71043=CARTESIAN_POINT('Ctrl Pts',(-18.5010374778185,-16.8477411199299,
-14.3011348233368));
#71044=CARTESIAN_POINT('Ctrl Pts',(-18.5230077067905,-16.8454247515293,
-14.2998398081182));
#71045=CARTESIAN_POINT('Ctrl Pts',(-18.730035253459,-16.8268688625312,-14.2877505853426));
#71046=CARTESIAN_POINT('Ctrl Pts',(-18.9164320929422,-16.8347086643427,
-14.2778149365771));
#71047=CARTESIAN_POINT('Ctrl Pts',(-19.2070661066051,-16.8856409444278,
-14.2617291744951));
#71048=CARTESIAN_POINT('Ctrl Pts',(-19.3130705856861,-16.912808455566,-14.2557044382252));
#71049=CARTESIAN_POINT('Ctrl Pts',(-19.4276556103934,-16.9518324946911,
-14.2485598568095));
#71050=CARTESIAN_POINT('Ctrl Pts',(-19.4387899194704,-16.9557286481411,
-14.2478587436266));
#71051=CARTESIAN_POINT('Ctrl Pts',(-19.4545994881612,-16.961409531765,-14.2468526484539));
#71052=CARTESIAN_POINT('Ctrl Pts',(-19.4593021097837,-16.9631181827622,
-14.2465520397536));
#71053=CARTESIAN_POINT('Ctrl Pts',(-19.4674061321594,-16.9660952631742,
-14.246031611518));
#71054=CARTESIAN_POINT('Ctrl Pts',(-19.4708104437233,-16.967355813172,-14.2458122610237));
#71055=CARTESIAN_POINT('Ctrl Pts',(-19.4774130277556,-16.9698199507624,
-14.2453853894602));
#71056=CARTESIAN_POINT('Ctrl Pts',(-19.4806116341742,-16.9710225279514,
-14.2451779346909));
#71057=CARTESIAN_POINT('Ctrl Pts',(-19.4892513653539,-16.9742946972862,
-14.244615827639));
#71058=CARTESIAN_POINT('Ctrl Pts',(-19.4946868407137,-16.9763789792127,
-14.2442603087065));
#71059=CARTESIAN_POINT('Ctrl Pts',(-19.5149313737947,-16.9842378586961,
-14.2429293226987));
#71060=CARTESIAN_POINT('Ctrl Pts',(-19.5296834171476,-16.9901566014415,
-14.241945734812));
#71061=CARTESIAN_POINT('Ctrl Pts',(-19.6585784742384,-17.0435641384826,
-14.233239633167));
#71062=CARTESIAN_POINT('Ctrl Pts',(-19.7684144681814,-17.1007966705077,
-14.2250589751229));
#71063=CARTESIAN_POINT('Ctrl Pts',(-20.0135263506943,-17.257173239253,-14.2058458527477));
#71064=CARTESIAN_POINT('Ctrl Pts',(-20.1433194170827,-17.3634582104785,
-14.1949293140074));
#71065=CARTESIAN_POINT('Ctrl Pts',(-20.2740377312084,-17.4992693764024,
-14.1833517784933));
#71066=CARTESIAN_POINT('Ctrl Pts',(-20.2885732311655,-17.5148345261482,
-14.1820538490488));
#71067=CARTESIAN_POINT('Ctrl Pts',(-20.3089101667041,-17.5372817067615,
-14.1802220646807));
#71068=CARTESIAN_POINT('Ctrl Pts',(-20.3149060430827,-17.5439850962232,
-14.1796799855965));
#71069=CARTESIAN_POINT('Ctrl Pts',(-20.3251770134136,-17.5556163612925,
-14.1787478162585));
#71070=CARTESIAN_POINT('Ctrl Pts',(-20.3294723460919,-17.5605261235653,
-14.1783568807515));
#71071=CARTESIAN_POINT('Ctrl Pts',(-20.3376538017579,-17.5699655929414,
-14.1776100974022));
#71072=CARTESIAN_POINT('Ctrl Pts',(-20.3415435918228,-17.5744920255406,
-14.1772540993608));
#71073=CARTESIAN_POINT('Ctrl Pts',(-20.3516099347434,-17.5863066360621,
-14.1763302980565));
#71074=CARTESIAN_POINT('Ctrl Pts',(-20.3577564321546,-17.5936203333132,
-14.1757637333954));
#71075=CARTESIAN_POINT('Ctrl Pts',(-20.3785534966147,-17.6187095625501,
-14.1738379040102));
#71076=CARTESIAN_POINT('Ctrl Pts',(-20.3929636857117,-17.6366828730015,
-14.1724883699118));
#71077=CARTESIAN_POINT('Ctrl Pts',(-20.514233751194,-17.793102936346,-14.1609878425405));
#71078=CARTESIAN_POINT('Ctrl Pts',(-20.6038500179196,-17.9440603936927,
-14.1515818059434));
#71079=CARTESIAN_POINT('Ctrl Pts',(-20.7088874074614,-18.184438461638,-14.1373097847421));
#71080=CARTESIAN_POINT('Ctrl Pts',(-20.7388925673333,-18.266628304272,-14.1325252852108));
#71081=CARTESIAN_POINT('Ctrl Pts',(-20.7745072694397,-18.386794187366,-14.1253702554482));
#71082=CARTESIAN_POINT('Ctrl Pts',(-20.7843049887495,-18.4234391443809,
-14.1231673023282));
#71083=CARTESIAN_POINT('Ctrl Pts',(-20.7948724745932,-18.4676952770427,
-14.1204601917538));
#71084=CARTESIAN_POINT('Ctrl Pts',(-20.7965927813452,-18.4750750209694,
-14.1200072372706));
#71085=CARTESIAN_POINT('Ctrl Pts',(-20.7992012880941,-18.4865430826915,
-14.1193007353718));
#71086=CARTESIAN_POINT('Ctrl Pts',(-20.8001170709358,-18.4906251516301,
-14.1190487424404));
#71087=CARTESIAN_POINT('Ctrl Pts',(-20.8017905239888,-18.4981894131817,
-14.118580793867));
#71088=CARTESIAN_POINT('Ctrl Pts',(-20.8025515038072,-18.5016708144893,
-14.1183650305685));
#71089=CARTESIAN_POINT('Ctrl Pts',(-20.8042489774775,-18.5095316647612,
-14.1178769641879));
#71090=CARTESIAN_POINT('Ctrl Pts',(-20.8051803614632,-18.5139121482261,
-14.1176043746306));
#71091=CARTESIAN_POINT('Ctrl Pts',(-20.807879766717,-18.5268090212333,-14.1168000903592));
#71092=CARTESIAN_POINT('Ctrl Pts',(-20.8096091841019,-18.5353332696965,
-14.1162662717741));
#71093=CARTESIAN_POINT('Ctrl Pts',(-20.8214936687642,-18.5958221781559,
-14.1124636819955));
#71094=CARTESIAN_POINT('Ctrl Pts',(-20.8297477350103,-18.6481367524029,
-14.1090992703783));
#71095=CARTESIAN_POINT('Ctrl Pts',(-20.8378088424033,-18.7155650890805,
-14.1047115704625));
#71096=CARTESIAN_POINT('Ctrl Pts',(-20.8394281570205,-18.7304478102423,
-14.1037399102944));
#71097=CARTESIAN_POINT('Ctrl Pts',(-20.8475637385171,-18.8133921847226,
-14.0983108221101));
#71098=CARTESIAN_POINT('Ctrl Pts',(-20.8509374103365,-18.8817197469213,
-14.0937882210587));
#71099=CARTESIAN_POINT('Ctrl Pts',(-20.8511442882195,-19.1108585921172,
-14.0786472789942));
#71100=CARTESIAN_POINT('Ctrl Pts',(-20.8329752262487,-19.2711508341196,
-14.0681492786479));
#71101=CARTESIAN_POINT('Ctrl Pts',(-20.7914795956747,-19.4510311537672,
-14.0567777760979));
#71102=CARTESIAN_POINT('Ctrl Pts',(-20.7857446847916,-19.4741093753488,
-14.0553254965786));
#71103=CARTESIAN_POINT('Ctrl Pts',(-20.7771304022459,-19.5064373723262,
-14.0532997977465));
#71104=CARTESIAN_POINT('Ctrl Pts',(-20.7745746985153,-19.515770826717,-14.0527159749718));
#71105=CARTESIAN_POINT('Ctrl Pts',(-20.7703333351151,-19.5308535536535,
-14.0517740932618));
#71106=CARTESIAN_POINT('Ctrl Pts',(-20.7686871312255,-19.5366136907826,
-14.0514147574334));
#71107=CARTESIAN_POINT('Ctrl Pts',(-20.7652024824747,-19.5486136004151,
-14.0506669103238));
#71108=CARTESIAN_POINT('Ctrl Pts',(-20.7633596820565,-19.5548520509312,
-14.0502785455249));
#71109=CARTESIAN_POINT('Ctrl Pts',(-20.7589304689817,-19.5695958416376,
-14.049361646217));
#71110=CARTESIAN_POINT('Ctrl Pts',(-20.7563191655654,-19.5780936224545,
-14.04883393154));
#71111=CARTESIAN_POINT('Ctrl Pts',(-20.7474528210905,-19.6063124414062,
-14.0470838497248));
#71112=CARTESIAN_POINT('Ctrl Pts',(-20.7409621030242,-19.6259586007358,
-14.0458692188294));
#71113=CARTESIAN_POINT('Ctrl Pts',(-20.7304048632613,-19.6564073564964,
-14.0439912770295));
#71114=CARTESIAN_POINT('Ctrl Pts',(-20.7265368266077,-19.6672754997887,
-14.0433218908956));
#71115=CARTESIAN_POINT('Ctrl Pts',(-20.7225805863163,-19.6781103578147,
-14.0426552896606));
#71116=CARTESIAN_POINT('Origin',(-18.734,-18.952,0.));
#71117=CARTESIAN_POINT('',(-20.7225805821191,-19.6781103693095,-13.2445592932782));
#71118=CARTESIAN_POINT('',(-20.7225805467356,-19.6781104662135,-13.4647889080502));
#71119=CARTESIAN_POINT('',(-20.7225805821191,-19.6781103693095,0.));
#71120=CARTESIAN_POINT('',(-20.8509991049198,-18.9539467328106,-13.5109437209775));
#71121=CARTESIAN_POINT('Ctrl Pts',(-20.7225805467356,-19.6781104662135,
-13.4647889080502));
#71122=CARTESIAN_POINT('Ctrl Pts',(-20.7382333305348,-19.635242579282,-13.4673503188061));
#71123=CARTESIAN_POINT('Ctrl Pts',(-20.7525027461134,-19.5918609102248,
-13.4699563619004));
#71124=CARTESIAN_POINT('Ctrl Pts',(-20.7697993275094,-19.5329117107744,
-13.4735579793603));
#71125=CARTESIAN_POINT('Ctrl Pts',(-20.7740668395333,-19.517742498761,-13.4744900743866));
#71126=CARTESIAN_POINT('Ctrl Pts',(-20.7796729213208,-19.4969265508334,
-13.4757781494082));
#71127=CARTESIAN_POINT('Ctrl Pts',(-20.7811583223091,-19.491319430789,-13.4761260033414));
#71128=CARTESIAN_POINT('Ctrl Pts',(-20.7834811071016,-19.4824034700739,
-13.476680645354));
#71129=CARTESIAN_POINT('Ctrl Pts',(-20.784333577585,-19.47909853887,-13.4768865675407));
#71130=CARTESIAN_POINT('Ctrl Pts',(-20.7860768719228,-19.4722717643364,
-13.4773126348401));
#71131=CARTESIAN_POINT('Ctrl Pts',(-20.7869666213465,-19.4687496956009,
-13.4775328428254));
#71132=CARTESIAN_POINT('Ctrl Pts',(-20.7890638347801,-19.4603569773869,
-13.4780584825616));
#71133=CARTESIAN_POINT('Ctrl Pts',(-20.7902630507495,-19.4554843060228,
-13.4783643854935));
#71134=CARTESIAN_POINT('Ctrl Pts',(-20.7927674028288,-19.4451503926449,
-13.4790146089627));
#71135=CARTESIAN_POINT('Ctrl Pts',(-20.7940681555771,-19.4396881395806,
-13.4793591675701));
#71136=CARTESIAN_POINT('Ctrl Pts',(-20.7975804740569,-19.424674048574,-13.4803085100425));
#71137=CARTESIAN_POINT('Ctrl Pts',(-20.7997474072569,-19.4151120495648,
-13.4809156168293));
#71138=CARTESIAN_POINT('Ctrl Pts',(-20.8343835369534,-19.2571922459627,
-13.4909794990141));
#71139=CARTESIAN_POINT('Ctrl Pts',(-20.8508585302458,-19.105796417632,-13.501135660806));
#71140=CARTESIAN_POINT('Ctrl Pts',(-20.850999092854,-18.9539598100794,-13.511142142957));
#71141=CARTESIAN_POINT('Ctrl Pts',(-20.8509991049198,-18.9539467328106,
-13.5109437209775));
#71142=CARTESIAN_POINT('Ctrl Pts',(-20.8510652701871,-18.8819944798437,
-13.5152699622426));
#71143=CARTESIAN_POINT('Ctrl Pts',(-20.84745892973,-18.8099473001284,-13.5195962035077));
#71144=CARTESIAN_POINT('Ctrl Pts',(-20.8401777557621,-18.7382144505981,
-13.5239224447729));
#71145=CARTESIAN_POINT('Ctrl Pts',(-20.8329012160598,-18.6665272570403,
-13.5282459325052));
#71146=CARTESIAN_POINT('Ctrl Pts',(-20.8219545300653,-18.59515448782,-13.5325694202375));
#71147=CARTESIAN_POINT('Ctrl Pts',(-20.8073873938027,-18.5245029646652,
-13.5368929079699));
#71148=CARTESIAN_POINT('Ctrl Pts',(-20.792824456527,-18.4538718068597,-13.541215149454));
#71149=CARTESIAN_POINT('Ctrl Pts',(-20.7746432396997,-18.3839619667449,
-13.545537390938));
#71150=CARTESIAN_POINT('Ctrl Pts',(-20.7529446959793,-18.3151708906015,
-13.5498596324221));
#71151=CARTESIAN_POINT('Ctrl Pts',(-20.7312448511874,-18.2463756896606,
-13.5541821330731));
#71152=CARTESIAN_POINT('Ctrl Pts',(-20.706027412668,-18.1786998565915,-13.5585046337241));
#71153=CARTESIAN_POINT('Ctrl Pts',(-20.67744287501,-18.1125246926962,-13.5628271343751));
#71154=CARTESIAN_POINT('Ctrl Pts',(-20.6488284904879,-18.0462804312647,
-13.5671541484134));
#71155=CARTESIAN_POINT('Ctrl Pts',(-20.6168401898347,-17.9815404195961,
-13.5714811624517));
#71156=CARTESIAN_POINT('Ctrl Pts',(-20.5816757716213,-17.9186640222254,
-13.57580817649));
#71157=CARTESIAN_POINT('Ctrl Pts',(-20.5464899011039,-17.8557492666601,
-13.5801378302541));
#71158=CARTESIAN_POINT('Ctrl Pts',(-20.5081243239348,-17.7947008039887,
-13.5844674840181));
#71159=CARTESIAN_POINT('Ctrl Pts',(-20.46682025899,-17.7358491252998,-13.5887971377822));
#71160=CARTESIAN_POINT('Ctrl Pts',(-20.4254474059601,-17.6768994346046,
-13.5931340021826));
#71161=CARTESIAN_POINT('Ctrl Pts',(-20.3811266092591,-17.6201542127691,
-13.597470866583));
#71162=CARTESIAN_POINT('Ctrl Pts',(-20.3341387764019,-17.5659102134945,
-13.6018077309834));
#71163=CARTESIAN_POINT('Ctrl Pts',(-20.3175654749946,-17.5467775552114,
-13.6033374069974));
#71164=CARTESIAN_POINT('Ctrl Pts',(-20.3006606978847,-17.5279557221356,
-13.6048670830114));
#71165=CARTESIAN_POINT('Ctrl Pts',(-20.2834377820478,-17.5094565657968,
-13.6063967590254));
#71166=CARTESIAN_POINT('Ctrl Pts',(-20.2340300954521,-17.4563877052551,
-13.6107849679563));
#71167=CARTESIAN_POINT('Ctrl Pts',(-20.1817963672775,-17.405756540934,-13.6151731768872));
#71168=CARTESIAN_POINT('Ctrl Pts',(-20.1270066890246,-17.3578791249304,
-13.6195613858181));
#71169=CARTESIAN_POINT('Ctrl Pts',(-20.0722983277386,-17.3100727669503,
-13.6239430819193));
#71170=CARTESIAN_POINT('Ctrl Pts',(-20.0150419071301,-17.2650123587827,
-13.6283247780206));
#71171=CARTESIAN_POINT('Ctrl Pts',(-19.9555455237308,-17.2229784462149,
-13.6327064741219));
#71172=CARTESIAN_POINT('Ctrl Pts',(-19.8961190533168,-17.1809939268396,
-13.6370830213815));
#71173=CARTESIAN_POINT('Ctrl Pts',(-19.8344582408823,-17.1420291152646,
-13.6414595686412));
#71174=CARTESIAN_POINT('Ctrl Pts',(-19.7709042257784,-17.1063243441593,
-13.6458361159008));
#71175=CARTESIAN_POINT('Ctrl Pts',(-19.7073905157072,-17.0706422165009,
-13.6502098876178));
#71176=CARTESIAN_POINT('Ctrl Pts',(-19.6419864047146,-17.0382162628698,
-13.6545836593348));
#71177=CARTESIAN_POINT('Ctrl Pts',(-19.5750607832521,-17.0092427431932,
-13.6589574310517));
#71178=CARTESIAN_POINT('Ctrl Pts',(-19.5081555274809,-16.980278040256,-13.6633298718153));
#71179=CARTESIAN_POINT('Ctrl Pts',(-19.4397301228477,-16.9547638770619,
-13.6677023125788));
#71180=CARTESIAN_POINT('Ctrl Pts',(-19.3701752330588,-16.9328491703583,
-13.6720747533424));
#71181=CARTESIAN_POINT('Ctrl Pts',(-19.3006185647437,-16.9109339032933,
-13.6764473059097));
#71182=CARTESIAN_POINT('Ctrl Pts',(-19.2299328146148,-16.8926184185036,
-13.6808198584771));
#71183=CARTESIAN_POINT('Ctrl Pts',(-19.1585240564096,-16.8780018501625,
-13.6851924110444));
#71184=CARTESIAN_POINT('Ctrl Pts',(-19.0870411875016,-16.8633701121954,
-13.6895695016118));
#71185=CARTESIAN_POINT('Ctrl Pts',(-19.0148342859533,-16.8524450521882,
-13.6939465921791));
#71186=CARTESIAN_POINT('Ctrl Pts',(-18.9423190546106,-16.8452745381787,
-13.6983236827464));
#71187=CARTESIAN_POINT('Ctrl Pts',(-18.8697642200086,-16.8381001080854,
-13.7027031638054));
#71188=CARTESIAN_POINT('Ctrl Pts',(-18.7969012025311,-16.8346843291133,
-13.7070826448643));
#71189=CARTESIAN_POINT('Ctrl Pts',(-18.7241475303631,-16.8350229267085,
-13.7114621259232));
#71190=CARTESIAN_POINT('Ctrl Pts',(-18.6512649027996,-16.8353621244656,
-13.715849369583));
#71191=CARTESIAN_POINT('Ctrl Pts',(-18.5784924896196,-16.839468960567,-13.7202366132427));
#71192=CARTESIAN_POINT('Ctrl Pts',(-18.5062439309009,-16.8472871518926,
-13.7246238569024));
#71193=CARTESIAN_POINT('Ctrl Pts',(-18.4571218728272,-16.8526027686348,
-13.7276067598372));
#71194=CARTESIAN_POINT('Ctrl Pts',(-18.4082418439352,-16.8596329436867,
-13.730589662772));
#71195=CARTESIAN_POINT('Ctrl Pts',(-18.3597305432932,-16.8683466282089,
-13.7335725657068));
#71196=CARTESIAN_POINT('Ctrl Pts',(-18.2883645862436,-16.8811655060194,
-13.7379607746377));
#71197=CARTESIAN_POINT('Ctrl Pts',(-18.217518663235,-16.8976801162965,-13.7423489835686));
#71198=CARTESIAN_POINT('Ctrl Pts',(-18.1476047194715,-16.9178344278368,
-13.7467371924995));
#71199=CARTESIAN_POINT('Ctrl Pts',(-18.0777945395923,-16.9379588270373,
-13.7511188886007));
#71200=CARTESIAN_POINT('Ctrl Pts',(-18.0089140527659,-16.9617120714412,
-13.755500584702));
#71201=CARTESIAN_POINT('Ctrl Pts',(-17.9413659204113,-16.9889869547365,
-13.7598822808033));
#71202=CARTESIAN_POINT('Ctrl Pts',(-17.873897162488,-17.0162297878734,-13.7642588280629));
#71203=CARTESIAN_POINT('Ctrl Pts',(-17.8077580939875,-17.0469858596163,
-13.7686353753226));
#71204=CARTESIAN_POINT('Ctrl Pts',(-17.7433354489119,-17.081098413273,-13.7730119225822));
#71205=CARTESIAN_POINT('Ctrl Pts',(-17.6789536597417,-17.115189333244,-13.7773856942992));
#71206=CARTESIAN_POINT('Ctrl Pts',(-17.6162865594632,-17.1526322864701,
-13.7817594660162));
#71207=CARTESIAN_POINT('Ctrl Pts',(-17.5556988450212,-17.1932233262362,
-13.7861332377332));
#71208=CARTESIAN_POINT('Ctrl Pts',(-17.4951295676243,-17.2338020140125,
-13.7905056784967));
#71209=CARTESIAN_POINT('Ctrl Pts',(-17.4366388203446,-17.2775266181314,
-13.7948781192603));
#71210=CARTESIAN_POINT('Ctrl Pts',(-17.3805632774546,-17.3241492580505,
-13.7992505600238));
#71211=CARTESIAN_POINT('Ctrl Pts',(-17.3244863007067,-17.3707730901158,
-13.8036231125912));
#71212=CARTESIAN_POINT('Ctrl Pts',(-17.2708250206033,-17.4202947951757,
-13.8079956651585));
#71213=CARTESIAN_POINT('Ctrl Pts',(-17.2198825933082,-17.4724265889274,
-13.8123682177259));
#71214=CARTESIAN_POINT('Ctrl Pts',(-17.1688872960406,-17.524612487021,-13.8167453082932));
#71215=CARTESIAN_POINT('Ctrl Pts',(-17.120616823207,-17.5794135364615,-13.8211223988605));
#71216=CARTESIAN_POINT('Ctrl Pts',(-17.0753364363177,-17.6365061070028,
-13.8254994894279));
#71217=CARTESIAN_POINT('Ctrl Pts',(-17.0300313201285,-17.693629857916,-13.8298789704868));
#71218=CARTESIAN_POINT('Ctrl Pts',(-16.9877198211676,-17.75304722842,-13.8342584515458));
#71219=CARTESIAN_POINT('Ctrl Pts',(-16.9486243452989,-17.8144048296514,
-13.8386379326047));
#71220=CARTESIAN_POINT('Ctrl Pts',(-16.9094595729617,-17.8758711868189,
-13.8430251762644));
#71221=CARTESIAN_POINT('Ctrl Pts',(-16.8735224451858,-17.9392842223086,
-13.8474124199242));
#71222=CARTESIAN_POINT('Ctrl Pts',(-16.8409895323028,-18.0042656652896,
-13.8517996635839));
#71223=CARTESIAN_POINT('Ctrl Pts',(-16.8188702864069,-18.0484467849189,
-13.8547825665187));
#71224=CARTESIAN_POINT('Ctrl Pts',(-16.7983237185202,-18.0933524542023,
-13.8577654694534));
#71225=CARTESIAN_POINT('Ctrl Pts',(-16.7793923012851,-18.1388593331259,
-13.8607483723882));
#71226=CARTESIAN_POINT('Ctrl Pts',(-16.7515419099038,-18.2058054245266,
-13.8651365813191));
#71227=CARTESIAN_POINT('Ctrl Pts',(-16.7270805292278,-18.2743146794849,
-13.86952479025));
#71228=CARTESIAN_POINT('Ctrl Pts',(-16.7061840240079,-18.3440103886485,
-13.8739129991809));
#71229=CARTESIAN_POINT('Ctrl Pts',(-16.6853185326665,-18.4136026578239,
-13.8782946952822));
#71230=CARTESIAN_POINT('Ctrl Pts',(-16.6680075510805,-18.4843774273511,
-13.8826763913834));
#71231=CARTESIAN_POINT('Ctrl Pts',(-16.6543788886961,-18.5559380939561,
-13.8870580874847));
#71232=CARTESIAN_POINT('Ctrl Pts',(-16.6407662410747,-18.6274146710828,
-13.8914346347443));
#71233=CARTESIAN_POINT('Ctrl Pts',(-16.6308274068039,-18.6996748392565,
-13.895811182004));
#71234=CARTESIAN_POINT('Ctrl Pts',(-16.6246399100932,-18.772308566959,-13.9001877292636));
#71235=CARTESIAN_POINT('Ctrl Pts',(-16.618456337403,-18.844896231407,-13.9045615009806));
#71236=CARTESIAN_POINT('Ctrl Pts',(-16.6160194227851,-18.917856505877,-13.9089352726976));
#71237=CARTESIAN_POINT('Ctrl Pts',(-16.6173550828665,-18.9907723454644,
-13.9133090444145));
#71238=CARTESIAN_POINT('Ctrl Pts',(-16.618690336502,-19.0636659965168,-13.9176814851781));
#71239=CARTESIAN_POINT('Ctrl Pts',(-16.6237958768595,-19.1365147575244,
-13.9220539259416));
#71240=CARTESIAN_POINT('Ctrl Pts',(-16.6326455110291,-19.2089013656677,
-13.9264263667052));
#71241=CARTESIAN_POINT('Ctrl Pts',(-16.6414953714849,-19.2812898247448,
-13.9307989192725));
#71242=CARTESIAN_POINT('Ctrl Pts',(-16.6540894553072,-19.3532156289256,
-13.9351714718399));
#71243=CARTESIAN_POINT('Ctrl Pts',(-16.6703498741219,-19.424268099667,-13.9395440244072));
#71244=CARTESIAN_POINT('Ctrl Pts',(-16.6866271686125,-19.4953943113425,
-13.9439211149746));
#71245=CARTESIAN_POINT('Ctrl Pts',(-16.7065782873148,-19.5656449087057,
-13.9482982055419));
#71246=CARTESIAN_POINT('Ctrl Pts',(-16.7300746894321,-19.6346216738906,
-13.9526752961092));
#71247=CARTESIAN_POINT('Ctrl Pts',(-16.7535839238067,-19.7036361098473,
-13.9570547771682));
#71248=CARTESIAN_POINT('Ctrl Pts',(-16.7806421175111,-19.7713748802477,
-13.9614342582271));
#71249=CARTESIAN_POINT('Ctrl Pts',(-16.8110725105123,-19.8374596942676,
-13.9658137392861));
#71250=CARTESIAN_POINT('Ctrl Pts',(-16.8415568411807,-19.9036616431767,
-13.9702009829458));
#71251=CARTESIAN_POINT('Ctrl Pts',(-16.8754250830335,-19.9682033538497,
-13.9745882266055));
#71252=CARTESIAN_POINT('Ctrl Pts',(-16.912454744336,-20.0307316077542,-13.9789754702652));
#71253=CARTESIAN_POINT('Ctrl Pts',(-16.9376313458521,-20.0732447952011,
-13.9819583732));
#71254=CARTESIAN_POINT('Ctrl Pts',(-16.9642684397431,-20.1148277943094,
-13.9849412761349));
#71255=CARTESIAN_POINT('Ctrl Pts',(-16.992285306212,-20.1553781306983,-13.9879241790697));
#71256=CARTESIAN_POINT('Ctrl Pts',(-17.033501486001,-20.2150325519721,-13.9923123880006));
#71257=CARTESIAN_POINT('Ctrl Pts',(-17.0778664461832,-20.2726834623514,
-13.9967005969315));
#71258=CARTESIAN_POINT('Ctrl Pts',(-17.1251586260628,-20.3279790817843,
-14.0010888058624));
#71259=CARTESIAN_POINT('Ctrl Pts',(-17.1723806165062,-20.3831926333497,
-14.0054705019636));
#71260=CARTESIAN_POINT('Ctrl Pts',(-17.2225208913247,-20.4360574697368,
-14.0098521980649));
#71261=CARTESIAN_POINT('Ctrl Pts',(-17.2753151507578,-20.4862514495973,
-14.0142338941662));
#71262=CARTESIAN_POINT('Ctrl Pts',(-17.3280473727347,-20.536386447537,-14.0186104414258));
#71263=CARTESIAN_POINT('Ctrl Pts',(-17.3834270362634,-20.583856492814,-14.0229869886854));
#71264=CARTESIAN_POINT('Ctrl Pts',(-17.4411513321102,-20.6283744575529,
-14.0273635359451));
#71265=CARTESIAN_POINT('Ctrl Pts',(-17.4988390200476,-20.6728641896455,
-14.031737307662));
#71266=CARTESIAN_POINT('Ctrl Pts',(-17.5588680090003,-20.7144052619587,
-14.036111079379));
#71267=CARTESIAN_POINT('Ctrl Pts',(-17.6209016583808,-20.7527501442134,
-14.040484851096));
#71268=CARTESIAN_POINT('Ctrl Pts',(-17.6829164307134,-20.7910833579916,
-14.0448572918595));
#71269=CARTESIAN_POINT('Ctrl Pts',(-17.7469342423156,-20.8262220591676,
-14.0492297326231));
#71270=CARTESIAN_POINT('Ctrl Pts',(-17.8125900634645,-20.8579624153833,
-14.0536021733866));
#71271=CARTESIAN_POINT('Ctrl Pts',(-17.8782475634398,-20.8897035832033,
-14.057974725954));
#71272=CARTESIAN_POINT('Ctrl Pts',(-17.9455427209576,-20.9180460253879,
-14.0623472785213));
#71273=CARTESIAN_POINT('Ctrl Pts',(-18.0140880608548,-20.9428329412274,
-14.0667198310886));
#71274=CARTESIAN_POINT('Ctrl Pts',(-18.0827045396913,-20.9676455818632,
-14.071096921656));
#71275=CARTESIAN_POINT('Ctrl Pts',(-18.1525733368264,-20.9888951643123,
-14.0754740122233));
#71276=CARTESIAN_POINT('Ctrl Pts',(-18.2232900373588,-21.0064742232647,
-14.0798511027906));
#71277=CARTESIAN_POINT('Ctrl Pts',(-18.2940453589062,-21.0240628827937,
-14.0842305838495));
#71278=CARTESIAN_POINT('Ctrl Pts',(-18.3656490319732,-21.0379769355906,
-14.0886100649085));
#71279=CARTESIAN_POINT('Ctrl Pts',(-18.4376872969889,-21.0481602472221,
-14.0929895459674));
#71280=CARTESIAN_POINT('Ctrl Pts',(-18.5098532493457,-21.0583616087051,
-14.0973767896272));
#71281=CARTESIAN_POINT('Ctrl Pts',(-18.5824548510274,-21.0648189809294,
-14.1017640332869));
#71282=CARTESIAN_POINT('Ctrl Pts',(-18.6550746705903,-21.0675282537413,
-14.1061512769466));
#71283=CARTESIAN_POINT('Ctrl Pts',(-18.7044491502641,-21.0693702981885,
-14.1091341798814));
#71284=CARTESIAN_POINT('Ctrl Pts',(-18.7538320255728,-21.069480806371,-14.1121170828162));
#71285=CARTESIAN_POINT('Ctrl Pts',(-18.8030934396838,-21.0678721834252,
-14.1150999857511));
#71286=CARTESIAN_POINT('Ctrl Pts',(-18.8755629038514,-21.0655057056244,
-14.119488194682));
#71287=CARTESIAN_POINT('Ctrl Pts',(-18.9480521075247,-21.0594071393707,
-14.1238764036129));
#71288=CARTESIAN_POINT('Ctrl Pts',(-19.020145332748,-21.0495723702763,-14.1282646125438));
#71289=CARTESIAN_POINT('Ctrl Pts',(-19.092131559672,-21.0397521976099,-14.132646308645));
#71290=CARTESIAN_POINT('Ctrl Pts',(-19.1637225008059,-21.0262068946333,
-14.1370280047463));
#71291=CARTESIAN_POINT('Ctrl Pts',(-19.2345042258083,-21.008984326617,-14.1414097008476));
#71292=CARTESIAN_POINT('Ctrl Pts',(-19.3052027766506,-20.9917819964888,
-14.1457862481073));
#71293=CARTESIAN_POINT('Ctrl Pts',(-19.3750935339407,-20.9709110986507,
-14.1501627953669));
#71294=CARTESIAN_POINT('Ctrl Pts',(-19.4437711636795,-20.9464708308745,
-14.1545393426265));
#71295=CARTESIAN_POINT('Ctrl Pts',(-19.5124052390636,-20.9220460627608,
-14.1589131143435));
#71296=CARTESIAN_POINT('Ctrl Pts',(-19.5798272600421,-20.8940565773994,
-14.1632868860605));
#71297=CARTESIAN_POINT('Ctrl Pts',(-19.6456468756575,-20.8626514528045,
-14.1676606577775));
#71298=CARTESIAN_POINT('Ctrl Pts',(-19.7114464621431,-20.8312558848944,
-14.172033098541));
#71299=CARTESIAN_POINT('Ctrl Pts',(-19.7756441762387,-20.7964469488634,
-14.1764055393046));
#71300=CARTESIAN_POINT('Ctrl Pts',(-19.8378710435228,-20.758421246352,-14.1807779800682));
#71301=CARTESIAN_POINT('Ctrl Pts',(-19.9000995019545,-20.7203945715193,
-14.1851505326355));
#71302=CARTESIAN_POINT('Ctrl Pts',(-19.9603566029539,-20.6791512201339,
-14.1895230852029));
#71303=CARTESIAN_POINT('Ctrl Pts',(-20.0183007689816,-20.6349321242383,
-14.1938956377702));
#71304=CARTESIAN_POINT('Ctrl Pts',(-20.0763050716505,-20.5906671360971,
-14.1982727283375));
#71305=CARTESIAN_POINT('Ctrl Pts',(-20.1319912623935,-20.5434205306327,
-14.2026498189049));
#71306=CARTESIAN_POINT('Ctrl Pts',(-20.185050077776,-20.493474187843,-14.2070269094722));
#71307=CARTESIAN_POINT('Ctrl Pts',(-20.2381378705468,-20.4435005675018,
-14.2114063905311));
#71308=CARTESIAN_POINT('Ctrl Pts',(-20.2885950971624,-20.3908246228575,
-14.2157858715901));
#71309=CARTESIAN_POINT('Ctrl Pts',(-20.3361505972396,-20.3357638757262,
-14.220165352649));
#71310=CARTESIAN_POINT('Ctrl Pts',(-20.3837903891216,-20.2806055337902,
-14.2245525963088));
#71311=CARTESIAN_POINT('Ctrl Pts',(-20.4285178872528,-20.2230543293395,
-14.2289398399685));
#71312=CARTESIAN_POINT('Ctrl Pts',(-20.4701036879215,-20.1634590314102,
-14.2333270836282));
#71313=CARTESIAN_POINT('Ctrl Pts',(-20.4983780251775,-20.1229399714081,
-14.236309986563));
#71314=CARTESIAN_POINT('Ctrl Pts',(-20.5252009588545,-20.0814766042671,
-14.2392928894977));
#71315=CARTESIAN_POINT('Ctrl Pts',(-20.5505126306684,-20.0391848336977,
-14.2422757924325));
#71316=CARTESIAN_POINT('Ctrl Pts',(-20.5890177730798,-19.9748488759396,
-14.2468135054349));
#71317=CARTESIAN_POINT('Ctrl Pts',(-20.6241652163778,-19.9083583182789,
-14.2513512184373));
#71318=CARTESIAN_POINT('Ctrl Pts',(-20.6557165770424,-19.8400846792511,
-14.2558889314397));
#71319=CARTESIAN_POINT('Ctrl Pts',(-20.6802004039359,-19.7871043980798,
-14.2594101925614));
#71320=CARTESIAN_POINT('Ctrl Pts',(-20.7025195175006,-19.7330511128152,
-14.262931453683));
#71321=CARTESIAN_POINT('Ctrl Pts',(-20.7225805821191,-19.6781103693095,
-14.2664527148047));
#71322=CARTESIAN_POINT('',(-20.8509999987353,-18.9520661441397,-13.2889079339059));
#71323=CARTESIAN_POINT('Ctrl Pts',(-20.7225805863163,-19.6781103578147,
-14.0426552896606));
#71324=CARTESIAN_POINT('Ctrl Pts',(-20.6958130594779,-19.7514179255168,
-14.0381451322549));
#71325=CARTESIAN_POINT('Ctrl Pts',(-20.6650078160421,-19.8232019799177,
-14.0337656063037));
#71326=CARTESIAN_POINT('Ctrl Pts',(-20.570357267885,-20.0139143494066,-14.0220205212262));
#71327=CARTESIAN_POINT('Ctrl Pts',(-20.4990150095605,-20.128686030151,-14.014842078084));
#71328=CARTESIAN_POINT('Ctrl Pts',(-20.3708542579152,-20.2967113021131,
-14.00314981442));
#71329=CARTESIAN_POINT('Ctrl Pts',(-20.3212057751213,-20.3549666842381,
-13.9988302312449));
#71330=CARTESIAN_POINT('Ctrl Pts',(-20.2619779473043,-20.4172858424494,
-13.9937348557344));
#71331=CARTESIAN_POINT('Ctrl Pts',(-20.2553888187653,-20.4241261026367,
-13.9931687258888));
#71332=CARTESIAN_POINT('Ctrl Pts',(-20.2455537548807,-20.4341994575187,
-13.9923243664036));
#71333=CARTESIAN_POINT('Ctrl Pts',(-20.2423428879629,-20.4374668347659,
-13.9920488096215));
#71334=CARTESIAN_POINT('Ctrl Pts',(-20.2366096482909,-20.443263223973,-13.9915569074305));
#71335=CARTESIAN_POINT('Ctrl Pts',(-20.2340914553369,-20.4457962992678,
-13.9913408910602));
#71336=CARTESIAN_POINT('Ctrl Pts',(-20.2286618086867,-20.4512304592593,
-13.9908751940785));
#71337=CARTESIAN_POINT('Ctrl Pts',(-20.2257483564714,-20.4541293994255,
-13.9906253579057));
#71338=CARTESIAN_POINT('Ctrl Pts',(-20.2176786545163,-20.4621122752175,
-13.989933542351));
#71339=CARTESIAN_POINT('Ctrl Pts',(-20.212504790597,-20.4671782120668,-13.9894901916504));
#71340=CARTESIAN_POINT('Ctrl Pts',(-20.1839451790823,-20.4948565043005,
-13.9870445508267));
#71341=CARTESIAN_POINT('Ctrl Pts',(-20.1600679645244,-20.5169527490522,
-13.98500593417));
#71342=CARTESIAN_POINT('Ctrl Pts',(-20.0137580935607,-20.6462202890972,
-13.9726000643451));
#71343=CARTESIAN_POINT('Ctrl Pts',(-19.8798138869347,-20.7395328337544,
-13.9616428011667));
#71344=CARTESIAN_POINT('Ctrl Pts',(-19.6336216829691,-20.8718996822781,
-13.9433847142914));
#71345=CARTESIAN_POINT('Ctrl Pts',(-19.5263234482218,-20.9186126517695,
-13.9359438713396));
#71346=CARTESIAN_POINT('Ctrl Pts',(-19.4021738934597,-20.9608396734241,
-13.9279368114988));
#71347=CARTESIAN_POINT('Ctrl Pts',(-19.388599174331,-20.9653040312148,-13.9270688353924));
#71348=CARTESIAN_POINT('Ctrl Pts',(-19.3669223587197,-20.9721905273076,
-13.9256945267389));
#71349=CARTESIAN_POINT('Ctrl Pts',(-19.3588493380864,-20.9747021003408,
-13.9251852661232));
#71350=CARTESIAN_POINT('Ctrl Pts',(-19.3445847676617,-20.9790463563296,
-13.9242898879908));
#71351=CARTESIAN_POINT('Ctrl Pts',(-19.3383995139578,-20.9808991887647,
-13.9239031143469));
#71352=CARTESIAN_POINT('Ctrl Pts',(-19.3255888931867,-20.9846729113781,
-13.9231050456488));
#71353=CARTESIAN_POINT('Ctrl Pts',(-19.3189624130423,-20.9865897768965,
-13.9226938859751));
#71354=CARTESIAN_POINT('Ctrl Pts',(-19.3019291080572,-20.9914269673407,
-13.9216411764047));
#71355=CARTESIAN_POINT('Ctrl Pts',(-19.2915089917432,-20.9943000655092,
-13.9210011678085));
#71356=CARTESIAN_POINT('Ctrl Pts',(-19.2479272897527,-21.0059582715653,
-13.9183405043392));
#71357=CARTESIAN_POINT('Ctrl Pts',(-19.2145755469596,-21.0140167750891,
-13.9163433781623));
#71358=CARTESIAN_POINT('Ctrl Pts',(-19.1271788951886,-21.0328978618357,
-13.9111993066022));
#71359=CARTESIAN_POINT('Ctrl Pts',(-19.0728803307786,-21.0424273060357,
-13.9080917500926));
#71360=CARTESIAN_POINT('Ctrl Pts',(-18.9099125740972,-21.0645104474783,
-13.8989473439218));
#71361=CARTESIAN_POINT('Ctrl Pts',(-18.8005787820791,-21.0707764803836,
-13.8930592236637));
#71362=CARTESIAN_POINT('Ctrl Pts',(-18.6455316024656,-21.0676449206137,
-13.8846160841683));
#71363=CARTESIAN_POINT('Ctrl Pts',(-18.599855691559,-21.0652404394081,-13.8821157478915));
#71364=CARTESIAN_POINT('Ctrl Pts',(-18.5315831001636,-21.0594240126794,
-13.8783162800304));
#71365=CARTESIAN_POINT('Ctrl Pts',(-18.5089045695325,-21.0571224586437,
-13.8770438075666));
#71366=CARTESIAN_POINT('Ctrl Pts',(-18.4852320985487,-21.0543331371715,
-13.8757007831837));
#71367=CARTESIAN_POINT('Ctrl Pts',(-18.4841960740489,-21.0542102861073,
-13.8756419760979));
#71368=CARTESIAN_POINT('Ctrl Pts',(-18.4647520122641,-21.0518900460502,
-13.8745377231388));
#71369=CARTESIAN_POINT('Ctrl Pts',(-18.4463740145589,-21.0494517730584,
-13.8734845244421));
#71370=CARTESIAN_POINT('Ctrl Pts',(-18.395068554122,-21.0419579355252,-13.8705119707729));
#71371=CARTESIAN_POINT('Ctrl Pts',(-18.3622264712923,-21.0363662975981,
-13.8685717292965));
#71372=CARTESIAN_POINT('Ctrl Pts',(-18.3227430090821,-21.0286811323164,
-13.8661790299478));
#71373=CARTESIAN_POINT('Ctrl Pts',(-18.3159605461909,-21.0273264441956,
-13.8657658562964));
#71374=CARTESIAN_POINT('Ctrl Pts',(-18.3048320049023,-21.0250469302752,
-13.8650842032775));
#71375=CARTESIAN_POINT('Ctrl Pts',(-18.3004819239325,-21.0241416023125,
-13.8648168120685));
#71376=CARTESIAN_POINT('Ctrl Pts',(-18.2926501571094,-21.0224859336363,
-13.864333666449));
#71377=CARTESIAN_POINT('Ctrl Pts',(-18.2891674908681,-21.021740496704,-13.8641181946151));
#71378=CARTESIAN_POINT('Ctrl Pts',(-18.2815707121067,-21.0200944069595,
-13.8636468100729));
#71379=CARTESIAN_POINT('Ctrl Pts',(-18.2774574516174,-21.0191902760618,
-13.863390704664));
#71380=CARTESIAN_POINT('Ctrl Pts',(-18.265824930441,-21.0165969333777,-13.8626640003407));
#71381=CARTESIAN_POINT('Ctrl Pts',(-18.2583122481092,-21.014878947389,-13.862191798882));
#71382=CARTESIAN_POINT('Ctrl Pts',(-18.2115906178136,-21.0039259414533,
-13.8592379839106));
#71383=CARTESIAN_POINT('Ctrl Pts',(-18.1726452438009,-20.9936150424382,
-13.8567004343362));
#71384=CARTESIAN_POINT('Ctrl Pts',(-17.9658344518386,-20.9324968498077,
-13.8429036509314));
#71385=CARTESIAN_POINT('Ctrl Pts',(-17.8044754330324,-20.862087847567,-13.8310594756206));
#71386=CARTESIAN_POINT('Ctrl Pts',(-17.6231896039867,-20.7545102229363,
-13.817408711854));
#71387=CARTESIAN_POINT('Ctrl Pts',(-17.5931950808407,-20.7356779892051,
-13.8151346568204));
#71388=CARTESIAN_POINT('Ctrl Pts',(-17.5108348252259,-20.6810397661047,
-13.8088525077503));
#71389=CARTESIAN_POINT('Ctrl Pts',(-17.4595822218534,-20.6436182244313,
-13.8048998612005));
#71390=CARTESIAN_POINT('Ctrl Pts',(-17.4003125151941,-20.5961178389879,
-13.8002730479109));
#71391=CARTESIAN_POINT('Ctrl Pts',(-17.3906115607842,-20.5882008701747,
-13.7995138155754));
#71392=CARTESIAN_POINT('Ctrl Pts',(-17.3748161558637,-20.5750750237738,
-13.7982742408212));
#71393=CARTESIAN_POINT('Ctrl Pts',(-17.3686801440415,-20.5699168546755,
-13.7977918571357));
#71394=CARTESIAN_POINT('Ctrl Pts',(-17.3577131987294,-20.5605907950322,
-13.7969281001716));
#71395=CARTESIAN_POINT('Ctrl Pts',(-17.3528715546427,-20.5564357026755,
-13.7965462090103));
#71396=CARTESIAN_POINT('Ctrl Pts',(-17.342612790318,-20.5475507973629,-13.7957357938495));
#71397=CARTESIAN_POINT('Ctrl Pts',(-17.3372008270287,-20.5428151327471,
-13.795307518859));
#71398=CARTESIAN_POINT('Ctrl Pts',(-17.3227223124671,-20.5300150574653,
-13.7941596766478));
#71399=CARTESIAN_POINT('Ctrl Pts',(-17.3137007039153,-20.5219000451298,
-13.7934422330006));
#71400=CARTESIAN_POINT('Ctrl Pts',(-17.2693543032314,-20.4813149060312,
-13.7899037184889));
#71401=CARTESIAN_POINT('Ctrl Pts',(-17.2350690976651,-20.4477265007838,
-13.7871307206324));
#71402=CARTESIAN_POINT('Ctrl Pts',(-17.0861946227446,-20.2916123914936,
-13.7748562278756));
#71403=CARTESIAN_POINT('Ctrl Pts',(-16.9852763364841,-20.1569029039112,
-13.7659337984802));
#71404=CARTESIAN_POINT('Ctrl Pts',(-16.8518811219019,-19.9262019060021,
-13.7513439704959));
#71405=CARTESIAN_POINT('Ctrl Pts',(-16.8084984036073,-19.837369583522,-13.7458494497216));
#71406=CARTESIAN_POINT('Ctrl Pts',(-16.7678421032428,-19.7368605735506,
-13.7394261789977));
#71407=CARTESIAN_POINT('Ctrl Pts',(-16.7642684258916,-19.7278482537088,
-13.7388484399939));
#71408=CARTESIAN_POINT('Ctrl Pts',(-16.7590835807036,-19.7145060504538,
-13.7379900563293));
#71409=CARTESIAN_POINT('Ctrl Pts',(-16.7574244231181,-19.7101947824483,
-13.7377122150107));
#71410=CARTESIAN_POINT('Ctrl Pts',(-16.7545060671554,-19.7025368449652,
-13.7372178024269));
#71411=CARTESIAN_POINT('Ctrl Pts',(-16.7532412227223,-19.6991923794091,
-13.7370015731437));
#71412=CARTESIAN_POINT('Ctrl Pts',(-16.7505494558862,-19.6920200182399,
-13.7365371924027));
#71413=CARTESIAN_POINT('Ctrl Pts',(-16.7491251598172,-19.688191249947,-13.736288894693));
#71414=CARTESIAN_POINT('Ctrl Pts',(-16.7452460607196,-19.677670434057,-13.7356055627893));
#71415=CARTESIAN_POINT('Ctrl Pts',(-16.7428139872269,-19.6709701447711,
-13.7351692110695));
#71416=CARTESIAN_POINT('Ctrl Pts',(-16.7300120784403,-19.6351380595596,
-13.7328299536195));
#71417=CARTESIAN_POINT('Ctrl Pts',(-16.7202482036132,-19.6057955854087,
-13.7308942755497));
#71418=CARTESIAN_POINT('Ctrl Pts',(-16.6926441574388,-19.516345496827,-13.7249549318184));
#71419=CARTESIAN_POINT('Ctrl Pts',(-16.6768287772441,-19.4556516428797,
-13.7208738366959));
#71420=CARTESIAN_POINT('Ctrl Pts',(-16.6356233923252,-19.2628039204623,
-13.7079148633303));
#71421=CARTESIAN_POINT('Ctrl Pts',(-16.62011557536,-19.1288652045959,-13.6989492342522));
#71422=CARTESIAN_POINT('Ctrl Pts',(-16.6166067523205,-18.9535302107213,
-13.6876558111758));
#71423=CARTESIAN_POINT('Ctrl Pts',(-16.6169711232901,-18.9126863708646,
-13.6850538712989));
#71424=CARTESIAN_POINT('Ctrl Pts',(-16.6203521445676,-18.8234178926193,
-13.6794348513671));
#71425=CARTESIAN_POINT('Ctrl Pts',(-16.6238520980651,-18.7750337559787,
-13.6764331910092));
#71426=CARTESIAN_POINT('Ctrl Pts',(-16.6303507814106,-18.7142867870322,
-13.672717270952));
#71427=CARTESIAN_POINT('Ctrl Pts',(-16.631802166116,-18.7017763311501,-13.6719547985169));
#71428=CARTESIAN_POINT('Ctrl Pts',(-16.6342793176457,-18.6819697761488,
-13.6707519229242));
#71429=CARTESIAN_POINT('Ctrl Pts',(-16.6352316620923,-18.6746649469813,
-13.6703092143439));
#71430=CARTESIAN_POINT('Ctrl Pts',(-16.6370774367705,-18.6610614634888,
-13.6694864484722));
#71431=CARTESIAN_POINT('Ctrl Pts',(-16.6379611641632,-18.6547615969657,
-13.6691060894844));
#71432=CARTESIAN_POINT('Ctrl Pts',(-16.639987347999,-18.6407759858801,-13.6682631452072));
#71433=CARTESIAN_POINT('Ctrl Pts',(-16.6411437520609,-18.6330923305548,
-13.6678010065479));
#71434=CARTESIAN_POINT('Ctrl Pts',(-16.6446277933629,-18.6107783101194,
-13.6664616348755));
#71435=CARTESIAN_POINT('Ctrl Pts',(-16.6470667570564,-18.5961656063579,
-13.6655879332183));
#71436=CARTESIAN_POINT('Ctrl Pts',(-16.6677249281885,-18.4799229437949,
-13.6586625321205));
#71437=CARTESIAN_POINT('Ctrl Pts',(-16.6932044991284,-18.3797175849504,
-13.6528538415446));
#71438=CARTESIAN_POINT('Ctrl Pts',(-16.7764326814558,-18.1303579151069,
-13.6383804516741));
#71439=CARTESIAN_POINT('Ctrl Pts',(-16.8439212937676,-17.9851700658453,
-13.6299536921691));
#71440=CARTESIAN_POINT('Ctrl Pts',(-16.9523809047564,-17.8074994601538,
-13.618198884059));
#71441=CARTESIAN_POINT('Ctrl Pts',(-16.9791052316602,-17.7669296862551,
-13.6154022716616));
#71442=CARTESIAN_POINT('Ctrl Pts',(-17.0116875206783,-17.7209886520113,
-13.6120585139978));
#71443=CARTESIAN_POINT('Ctrl Pts',(-17.0162112748365,-17.7146839098953,
-13.6115956410275));
#71444=CARTESIAN_POINT('Ctrl Pts',(-17.0234999390514,-17.7046427352062,
-13.6108517977022));
#71445=CARTESIAN_POINT('Ctrl Pts',(-17.0262427189144,-17.7008902236435,
-13.6105723151012));
#71446=CARTESIAN_POINT('Ctrl Pts',(-17.0311248243385,-17.694256777935,-13.610075542032));
#71447=CARTESIAN_POINT('Ctrl Pts',(-17.0332591429314,-17.691372214542,-13.609858600215));
#71448=CARTESIAN_POINT('Ctrl Pts',(-17.0378013193579,-17.6852659266808,
-13.6093973848977));
#71449=CARTESIAN_POINT('Ctrl Pts',(-17.0402109897701,-17.6820456839236,
-13.6091529891958));
#71450=CARTESIAN_POINT('Ctrl Pts',(-17.0467453190594,-17.6733649968834,
-13.608491066855));
#71451=CARTESIAN_POINT('Ctrl Pts',(-17.050887260276,-17.667917708255,-13.6080723543029));
#71452=CARTESIAN_POINT('Ctrl Pts',(-17.0716513221643,-17.6408828449773,
-13.6059779703024));
#71453=CARTESIAN_POINT('Ctrl Pts',(-17.0886618705169,-17.619598559898,-13.6042769863701));
#71454=CARTESIAN_POINT('Ctrl Pts',(-17.1391486009376,-17.5588689130347,
-13.599284761692));
#71455=CARTESIAN_POINT('Ctrl Pts',(-17.1736646918612,-17.5203163000448,
-13.5959403877277));
#71456=CARTESIAN_POINT('Ctrl Pts',(-17.3054203723514,-17.3835813132554,
-13.5835285051363));
#71457=CARTESIAN_POINT('Ctrl Pts',(-17.4108030784123,-17.2937084497809,
-13.5742897737105));
#71458=CARTESIAN_POINT('Ctrl Pts',(-17.6031704743741,-17.1597454553624,
-13.5591100729883));
#71459=CARTESIAN_POINT('Ctrl Pts',(-17.6858164728997,-17.1101890588021,
-13.5530293088708));
#71460=CARTESIAN_POINT('Ctrl Pts',(-17.7839415884109,-17.06010378842,-13.5463058347475));
#71461=CARTESIAN_POINT('Ctrl Pts',(-17.7963858895196,-17.0539056780228,
-13.5454617093154));
#71462=CARTESIAN_POINT('Ctrl Pts',(-17.8163935981916,-17.0441852620685,
-13.5441179456696));
#71463=CARTESIAN_POINT('Ctrl Pts',(-17.8239181787173,-17.0405843820378,
-13.5436155784605));
#71464=CARTESIAN_POINT('Ctrl Pts',(-17.8372882116439,-17.0342830172411,
-13.5427281878522));
#71465=CARTESIAN_POINT('Ctrl Pts',(-17.8431250340579,-17.0315645666108,
-13.5423425451855));
#71466=CARTESIAN_POINT('Ctrl Pts',(-17.8552841475793,-17.0259689259553,
-13.5415427900568));
#71467=CARTESIAN_POINT('Ctrl Pts',(-17.8616083869506,-17.0230961343992,
-13.5411288328822));
#71468=CARTESIAN_POINT('Ctrl Pts',(-17.878008453911,-17.0157435447766,-13.5400604892632));
#71469=CARTESIAN_POINT('Ctrl Pts',(-17.8881054288738,-17.0113112127731,
-13.5394077349168));
#71470=CARTESIAN_POINT('Ctrl Pts',(-17.9315449037819,-16.9926457462694,
-13.536620257447));
#71471=CARTESIAN_POINT('Ctrl Pts',(-17.9652165596594,-16.9791909556015,
-13.5345120219859));
#71472=CARTESIAN_POINT('Ctrl Pts',(-18.055007263207,-16.9459599898318,-13.5290129268166));
#71473=CARTESIAN_POINT('Ctrl Pts',(-18.1116438435915,-16.9276726411516,
-13.5256689800554));
#71474=CARTESIAN_POINT('Ctrl Pts',(-18.3313423076377,-16.8668286551017,
-13.5130362316837));
#71475=CARTESIAN_POINT('Ctrl Pts',(-18.4984768940598,-16.8414091189746,
-13.5041712361617));
#71476=CARTESIAN_POINT('Ctrl Pts',(-18.7205483698113,-16.8343609538018,
-13.4916799741708));
#71477=CARTESIAN_POINT('Ctrl Pts',(-18.7742935543018,-16.8347018474999,
-13.4885976398515));
#71478=CARTESIAN_POINT('Ctrl Pts',(-18.8366877340728,-16.8374739278206,
-13.4848914337852));
#71479=CARTESIAN_POINT('Ctrl Pts',(-18.8454103542768,-16.837915562786,-13.4843703969722));
#71480=CARTESIAN_POINT('Ctrl Pts',(-18.8586087614712,-16.8386657192304,
-13.4835772560194));
#71481=CARTESIAN_POINT('Ctrl Pts',(-18.8630868338411,-16.83893452203,-13.4833073242564));
#71482=CARTESIAN_POINT('Ctrl Pts',(-18.871121040528,-16.8394424212446,-13.4828214941084));
#71483=CARTESIAN_POINT('Ctrl Pts',(-18.8746774529178,-16.8396762659908,
-13.4826058928054));
#71484=CARTESIAN_POINT('Ctrl Pts',(-18.8824012148666,-16.840203719118,-13.482136458809));
#71485=CARTESIAN_POINT('Ctrl Pts',(-18.8865682360268,-16.8405006783851,
-13.481882445683));
#71486=CARTESIAN_POINT('Ctrl Pts',(-18.8982638989283,-16.8413689619674,
-13.4811674471303));
#71487=CARTESIAN_POINT('Ctrl Pts',(-18.9057903147636,-16.8419682251193,
-13.48070493855));
#71488=CARTESIAN_POINT('Ctrl Pts',(-18.9506294209084,-16.84577986564,-13.4779359039066));
#71489=CARTESIAN_POINT('Ctrl Pts',(-18.987852292974,-16.8499414435024,-13.4755810765705));
#71490=CARTESIAN_POINT('Ctrl Pts',(-19.1096723722018,-16.8668437378152,
-13.4677314366213));
#71491=CARTESIAN_POINT('Ctrl Pts',(-19.1936065901604,-16.8837238401075,
-13.4620980916345));
#71492=CARTESIAN_POINT('Ctrl Pts',(-19.4479091261381,-16.9511135519632,
-13.4447180654062));
#71493=CARTESIAN_POINT('Ctrl Pts',(-19.6131680269204,-17.0180143043342,
-13.4330524665178));
#71494=CARTESIAN_POINT('Ctrl Pts',(-19.7880620718266,-17.1159273293674,
-13.4207171625239));
#71495=CARTESIAN_POINT('Ctrl Pts',(-19.8077921083987,-17.1273958579983,
-13.4193242841738));
#71496=CARTESIAN_POINT('Ctrl Pts',(-19.8353271342834,-17.1440025762275,
-13.4173778475465));
#71497=CARTESIAN_POINT('Ctrl Pts',(-19.8432889032704,-17.1488765226628,
-13.4168147248669));
#71498=CARTESIAN_POINT('Ctrl Pts',(-19.8567579545737,-17.1572448329992,
-13.4158614725421));
#71499=CARTESIAN_POINT('Ctrl Pts',(-19.862281747963,-17.160712241786,-13.4154703583744));
#71500=CARTESIAN_POINT('Ctrl Pts',(-19.8732383562729,-17.1676607388309,
-13.4146941837743));
#71501=CARTESIAN_POINT('Ctrl Pts',(-19.8786714536052,-17.1711412475788,
-13.41430910749));
#71502=CARTESIAN_POINT('Ctrl Pts',(-19.8895652008054,-17.1781903658174,
-13.413536575524));
#71503=CARTESIAN_POINT('Ctrl Pts',(-19.8950254385381,-17.181759484095,-13.4131491443765));
#71504=CARTESIAN_POINT('Ctrl Pts',(-19.9145651278664,-17.1946610173911,
-13.4117618411988));
#71505=CARTESIAN_POINT('Ctrl Pts',(-19.9285495108308,-17.2041367869009,
-13.4107673469734));
#71506=CARTESIAN_POINT('Ctrl Pts',(-20.0547616540925,-17.2918800599656,
-13.4017728488539));
#71507=CARTESIAN_POINT('Ctrl Pts',(-20.1592737051247,-17.3806911619782,
-13.394216406992));
#71508=CARTESIAN_POINT('Ctrl Pts',(-20.3678976506755,-17.5960388531668,
-13.3778937736117));
#71509=CARTESIAN_POINT('Ctrl Pts',(-20.4673865506338,-17.7257835060041,
-13.3692248150557));
#71510=CARTESIAN_POINT('Ctrl Pts',(-20.5582171469079,-17.8777008255907,
-13.3588209721347));
#71511=CARTESIAN_POINT('Ctrl Pts',(-20.5653157397344,-17.8898467375748,
-13.3579873443408));
#71512=CARTESIAN_POINT('Ctrl Pts',(-20.575038350056,-17.9068696514844,-13.3568151589996));
#71513=CARTESIAN_POINT('Ctrl Pts',(-20.5777652552586,-17.9116878671795,
-13.3564829572085));
#71514=CARTESIAN_POINT('Ctrl Pts',(-20.5821176096883,-17.9194489826807,
-13.3559470820917));
#71515=CARTESIAN_POINT('Ctrl Pts',(-20.5837550245248,-17.9223851926633,
-13.3557441720481));
#71516=CARTESIAN_POINT('Ctrl Pts',(-20.5871657415607,-17.9285356818154,
-13.3553187414431));
#71517=CARTESIAN_POINT('Ctrl Pts',(-20.5889376786719,-17.931750675663,-13.3550961329588));
#71518=CARTESIAN_POINT('Ctrl Pts',(-20.5932122404427,-17.9395543646391,
-13.3545552800165));
#71519=CARTESIAN_POINT('Ctrl Pts',(-20.5957062415976,-17.9441477349192,
-13.3542364919918));
#71520=CARTESIAN_POINT('Ctrl Pts',(-20.6044137014452,-17.9603274548222,
-13.3531121965151));
#71521=CARTESIAN_POINT('Ctrl Pts',(-20.6105360659002,-17.9719621309205,
-13.3523012230678));
#71522=CARTESIAN_POINT('Ctrl Pts',(-20.6463529977379,-18.0415932943318,
-13.3474362625599));
#71523=CARTESIAN_POINT('Ctrl Pts',(-20.673462968082,-18.1008736150483,-13.3432483730028));
#71524=CARTESIAN_POINT('Ctrl Pts',(-20.7663306087012,-18.3315219542664,
-13.3270239402859));
#71525=CARTESIAN_POINT('Ctrl Pts',(-20.8124570528268,-18.5099651622943,
-13.3147003989581));
#71526=CARTESIAN_POINT('Ctrl Pts',(-20.8382409111785,-18.718416868344,-13.3013963293275));
#71527=CARTESIAN_POINT('Ctrl Pts',(-20.8409993885486,-18.7447693006873,
-13.2997318868771));
#71528=CARTESIAN_POINT('Ctrl Pts',(-20.8463154969658,-18.8067773330992,
-13.295856603968));
#71529=CARTESIAN_POINT('Ctrl Pts',(-20.848466290051,-18.8424603529987,-13.2936584702531));
#71530=CARTESIAN_POINT('Ctrl Pts',(-20.8501018468728,-18.8893377032315,
-13.2908108478712));
#71531=CARTESIAN_POINT('Ctrl Pts',(-20.8504028282094,-18.9004959613303,
-13.2901359888879));
#71532=CARTESIAN_POINT('Ctrl Pts',(-20.8507477576331,-18.9185925177508,
-13.2890461762796));
#71533=CARTESIAN_POINT('Ctrl Pts',(-20.8508458709918,-18.9255294585662,
-13.2886295333159));
#71534=CARTESIAN_POINT('Ctrl Pts',(-20.8509497984574,-18.9367926063628,
-13.2879548253289));
#71535=CARTESIAN_POINT('Ctrl Pts',(-20.8509764542885,-18.9411185282282,
-13.2876961097797));
#71536=CARTESIAN_POINT('Ctrl Pts',(-20.8509965706207,-18.947614789788,-13.2873082240935));
#71537=CARTESIAN_POINT('Ctrl Pts',(-20.8509999537562,-18.9497850671378,
-13.2871787442691));
#71538=CARTESIAN_POINT('Ctrl Pts',(-20.8509999995292,-18.9519553508202,
-13.2870493686989));
#71539=CARTESIAN_POINT('Ctrl Pts',(-20.8509999986719,-18.9520749873283,
-13.2890562789747));
#71540=CARTESIAN_POINT('Ctrl Pts',(-20.8509972774554,-19.0288988399363,
-13.2844612169094));
#71541=CARTESIAN_POINT('Ctrl Pts',(-20.846808461958,-19.1056371709782,-13.2798661548441));
#71542=CARTESIAN_POINT('Ctrl Pts',(-20.8384871131054,-19.181832527666,-13.2752710927788));
#71543=CARTESIAN_POINT('Ctrl Pts',(-20.8301538008358,-19.258137428713,-13.2706694244956));
#71544=CARTESIAN_POINT('Ctrl Pts',(-20.8176761741826,-19.3338973982161,
-13.2660677562124));
#71545=CARTESIAN_POINT('Ctrl Pts',(-20.8011589270257,-19.408665052766,-13.2614660879292));
#71546=CARTESIAN_POINT('Ctrl Pts',(-20.784602739877,-19.4836089746948,-13.256853571051));
#71547=CARTESIAN_POINT('Ctrl Pts',(-20.7639880126746,-19.5575555158826,
-13.2522410541727));
#71548=CARTESIAN_POINT('Ctrl Pts',(-20.7394693418677,-19.6300720602036,
-13.2476285372945));
#71549=CARTESIAN_POINT('Ctrl Pts',(-20.7340309672849,-19.6461566242721,
-13.2466054559557));
#71550=CARTESIAN_POINT('Ctrl Pts',(-20.728400713704,-19.6621709183055,-13.245582374617));
#71551=CARTESIAN_POINT('Ctrl Pts',(-20.7225805821191,-19.6781103693095,
-13.2445592932782));
#71552=CARTESIAN_POINT('Origin',(-18.734,-18.952,0.));
#71553=CARTESIAN_POINT('',(-20.7242504220745,-19.678735851896,-12.4443820803097));
#71554=CARTESIAN_POINT('',(-20.7225804971235,-19.678110602085,-12.6679319461521));
#71555=CARTESIAN_POINT('',(-20.7225805821191,-19.6781103693095,0.));
#71556=CARTESIAN_POINT('Ctrl Pts',(-20.7225804971235,-19.6781106020849,
-12.6679319461521));
#71557=CARTESIAN_POINT('Ctrl Pts',(-20.7627960942047,-19.5679731770063,
-12.6745736078838));
#71558=CARTESIAN_POINT('Ctrl Pts',(-20.7938156866259,-19.4546218238198,
-12.6809438939));
#71559=CARTESIAN_POINT('Ctrl Pts',(-20.8390879830612,-19.2112808287383,
-12.694385289415));
#71560=CARTESIAN_POINT('Ctrl Pts',(-20.8510398086386,-19.0814434490627,
-12.7014276962788));
#71561=CARTESIAN_POINT('Ctrl Pts',(-20.8509988957479,-18.948075646787,-12.709218677413));
#71562=CARTESIAN_POINT('Ctrl Pts',(-20.8509902918148,-18.9448007475233,
-12.7094103387302));
#71563=CARTESIAN_POINT('Ctrl Pts',(-20.850896614057,-18.925867051309,-12.7105205155376));
#71564=CARTESIAN_POINT('Ctrl Pts',(-20.8506454058121,-18.9102100571119,
-12.7114468464764));
#71565=CARTESIAN_POINT('Ctrl Pts',(-20.8500635609687,-18.8887743830472,
-12.7127281576504));
#71566=CARTESIAN_POINT('Ctrl Pts',(-20.8498828713514,-18.882991698817,-12.7130751213308));
#71567=CARTESIAN_POINT('Ctrl Pts',(-20.8495580067021,-18.873801856879,-12.7136286934075));
#71568=CARTESIAN_POINT('Ctrl Pts',(-20.8494292971625,-18.8703941323496,
-12.7138344418728));
#71569=CARTESIAN_POINT('Ctrl Pts',(-20.8491463981908,-18.8633550635714,
-12.7142604510224));
#71570=CARTESIAN_POINT('Ctrl Pts',(-20.8489910909365,-18.859723811226,-12.7144807759306));
#71571=CARTESIAN_POINT('Ctrl Pts',(-20.8485986130547,-18.8510693566604,
-12.7150071901784));
#71572=CARTESIAN_POINT('Ctrl Pts',(-20.8483528940849,-18.846046580164,-12.7153137543883));
#71573=CARTESIAN_POINT('Ctrl Pts',(-20.8474631299072,-18.8290964806147,
-12.716351735142));
#71574=CARTESIAN_POINT('Ctrl Pts',(-20.8467360486436,-18.8171740001958,
-12.7170875791991));
#71575=CARTESIAN_POINT('Ctrl Pts',(-20.8368861065989,-18.6754132077932,
-12.7259001726146));
#71576=CARTESIAN_POINT('Ctrl Pts',(-20.8159094459839,-18.5466897737048,
-12.7345169939419));
#71577=CARTESIAN_POINT('Ctrl Pts',(-20.742511607016,-18.2635785876856,-12.7538436953377));
#71578=CARTESIAN_POINT('Ctrl Pts',(-20.68382371734,-18.1116136822067,-12.7644503905451));
#71579=CARTESIAN_POINT('Ctrl Pts',(-20.5973010332701,-17.9468329361202,
-12.7759142878588));
#71580=CARTESIAN_POINT('Ctrl Pts',(-20.5859221280117,-17.9260194590116,
-12.7773628960543));
#71581=CARTESIAN_POINT('Ctrl Pts',(-20.5694163735905,-17.8969980170267,
-12.7793843750634));
#71582=CARTESIAN_POINT('Ctrl Pts',(-20.5645797181732,-17.8886278408834,
-12.7799675916828));
#71583=CARTESIAN_POINT('Ctrl Pts',(-20.5566540403871,-17.8751262304901,
-12.7809087582783));
#71584=CARTESIAN_POINT('Ctrl Pts',(-20.5536003185196,-17.8699743309944,
-12.7812679813822));
#71585=CARTESIAN_POINT('Ctrl Pts',(-20.5471835197496,-17.8592526114134,
-12.782015798378));
#71586=CARTESIAN_POINT('Ctrl Pts',(-20.5438165410143,-17.8536851904471,
-12.7824042448905));
#71587=CARTESIAN_POINT('Ctrl Pts',(-20.5357843190278,-17.8405408512395,
-12.7833217022563));
#71588=CARTESIAN_POINT('Ctrl Pts',(-20.5310968440375,-17.832977610371,-12.7838498904967));
#71589=CARTESIAN_POINT('Ctrl Pts',(-20.5153272651458,-17.8078880526529,
-12.7856031948381));
#71590=CARTESIAN_POINT('Ctrl Pts',(-20.5040351435845,-17.7904946796791,
-12.7868205349196));
#71591=CARTESIAN_POINT('Ctrl Pts',(-20.442391612741,-17.6985317796352,-12.7932716438279));
#71592=CARTESIAN_POINT('Ctrl Pts',(-20.3875775967268,-17.6270591357007,
-12.7983324571827));
#71593=CARTESIAN_POINT('Ctrl Pts',(-20.239226675372,-17.4572274408571,-12.8107698012182));
#71594=CARTESIAN_POINT('Ctrl Pts',(-20.1404888688135,-17.3639700355569,
-12.8179823280751));
#71595=CARTESIAN_POINT('Ctrl Pts',(-19.9740075103769,-17.234515345521,-12.8296580700672));
#71596=CARTESIAN_POINT('Ctrl Pts',(-19.9120725274929,-17.1914561278076,
-12.833918237911));
#71597=CARTESIAN_POINT('Ctrl Pts',(-19.8399118466703,-17.1468024930102,
-12.8389476021337));
#71598=CARTESIAN_POINT('Ctrl Pts',(-19.8318090219815,-17.1418634318041,
-12.8395132495199));
#71599=CARTESIAN_POINT('Ctrl Pts',(-19.8197472544567,-17.1346219792095,
-12.8403570256971));
#71600=CARTESIAN_POINT('Ctrl Pts',(-19.8158134764321,-17.1322776111949,
-12.8406324869893));
#71601=CARTESIAN_POINT('Ctrl Pts',(-19.8087980622483,-17.1281275037412,
-12.8411242847666));
#71602=CARTESIAN_POINT('Ctrl Pts',(-19.8057194325292,-17.126316781331,-12.8413402927544));
#71603=CARTESIAN_POINT('Ctrl Pts',(-19.7990873153699,-17.1224386012612,
-12.8418060471112));
#71604=CARTESIAN_POINT('Ctrl Pts',(-19.795532435717,-17.1203737312504,-12.8420559494402));
#71605=CARTESIAN_POINT('Ctrl Pts',(-19.7856953558016,-17.1146980697889,
-12.8427481304321));
#71606=CARTESIAN_POINT('Ctrl Pts',(-19.7794006661124,-17.1111091971637,
-12.8431917827522));
#71607=CARTESIAN_POINT('Ctrl Pts',(-19.7446834628047,-17.0915509136805,
-12.8456421382928));
#71608=CARTESIAN_POINT('Ctrl Pts',(-19.7159150516618,-17.0762083203526,
-12.8476853299662));
#71609=CARTESIAN_POINT('Ctrl Pts',(-19.5415619113382,-16.9883331863171,
-12.8600927436671));
#71610=CARTESIAN_POINT('Ctrl Pts',(-19.3883700340201,-16.9321130246887,
-12.871045822317));
#71611=CARTESIAN_POINT('Ctrl Pts',(-19.1167156872076,-16.8666084178378,
-12.8892985597815));
#71612=CARTESIAN_POINT('Ctrl Pts',(-19.001093166878,-16.8486696905022,-12.8967380863076));
#71613=CARTESIAN_POINT('Ctrl Pts',(-18.8703108069129,-16.8393446703619,
-12.904743920682));
#71614=CARTESIAN_POINT('Ctrl Pts',(-18.8560477180726,-16.8384727235829,
-12.9056118806448));
#71615=CARTESIAN_POINT('Ctrl Pts',(-18.833333140478,-16.8373148213725,-12.9069861686449));
#71616=CARTESIAN_POINT('Ctrl Pts',(-18.8248870704841,-16.8369349841761,
-12.9074954246141));
#71617=CARTESIAN_POINT('Ctrl Pts',(-18.8099870466371,-16.836354316576,-12.9083907973364));
#71618=CARTESIAN_POINT('Ctrl Pts',(-18.80353406734,-16.8361323992369,-12.9087775701918));
#71619=CARTESIAN_POINT('Ctrl Pts',(-18.7901850928668,-16.8357344639777,
-12.9095756399051));
#71620=CARTESIAN_POINT('Ctrl Pts',(-18.7832890427834,-16.835562621855,-12.9099868013696));
#71621=CARTESIAN_POINT('Ctrl Pts',(-18.7655855904696,-16.8352080450825,
-12.9110395209943));
#71622=CARTESIAN_POINT('Ctrl Pts',(-18.7547773213561,-16.8350743661137,
-12.9116795377962));
#71623=CARTESIAN_POINT('Ctrl Pts',(-18.7096623972587,-16.8348619304664,
-12.9143402810845));
#71624=CARTESIAN_POINT('Ctrl Pts',(-18.675356274072,-16.8355343058755,-12.9163374770723));
#71625=CARTESIAN_POINT('Ctrl Pts',(-18.586025601785,-16.8394590109449,-12.9214817691025));
#71626=CARTESIAN_POINT('Ctrl Pts',(-18.5310840017961,-16.8440266614322,
-12.9245894718428));
#71627=CARTESIAN_POINT('Ctrl Pts',(-18.3678441800644,-16.8640402229597,
-12.9337341331152));
#71628=CARTESIAN_POINT('Ctrl Pts',(-18.2604994115583,-16.8857366597852,
-12.9396223630923));
#71629=CARTESIAN_POINT('Ctrl Pts',(-18.1111156439335,-16.9281879776657,
-12.9480774751203));
#71630=CARTESIAN_POINT('Ctrl Pts',(-18.0673414866058,-16.9421825436189,
-12.9505897536701));
#71631=CARTESIAN_POINT('Ctrl Pts',(-18.0030660994603,-16.9650623657529,
-12.9543734436541));
#71632=CARTESIAN_POINT('Ctrl Pts',(-17.9821932981216,-16.9728658044634,
-12.9556173912177));
#71633=CARTESIAN_POINT('Ctrl Pts',(-17.9135904234385,-16.9997553035697,
-12.9597681002729));
#71634=CARTESIAN_POINT('Ctrl Pts',(-17.8664359112616,-17.020248758664,-12.962721747538));
#71635=CARTESIAN_POINT('Ctrl Pts',(-17.8129726159367,-17.045836415554,-12.9662396599061));
#71636=CARTESIAN_POINT('Ctrl Pts',(-17.8058862825645,-17.0492766948379,
-12.9667094508007));
#71637=CARTESIAN_POINT('Ctrl Pts',(-17.7946186733942,-17.0548248240846,
-12.9674623054615));
#71638=CARTESIAN_POINT('Ctrl Pts',(-17.7904248276733,-17.0569071742813,
-12.9677438240295));
#71639=CARTESIAN_POINT('Ctrl Pts',(-17.783025069199,-17.0606119934541,-12.9682429119953));
#71640=CARTESIAN_POINT('Ctrl Pts',(-17.7798163357228,-17.0622287320972,
-12.9684601214531));
#71641=CARTESIAN_POINT('Ctrl Pts',(-17.773041272701,-17.0656640411195,-12.9689204449763));
#71642=CARTESIAN_POINT('Ctrl Pts',(-17.7694760366275,-17.067484532087,-12.9691636739118));
#71643=CARTESIAN_POINT('Ctrl Pts',(-17.7599056496108,-17.0724056627488,
-12.9698192185863));
#71644=CARTESIAN_POINT('Ctrl Pts',(-17.7539102068058,-17.0755249347479,
-12.9702326821631));
#71645=CARTESIAN_POINT('Ctrl Pts',(-17.7247069458194,-17.0908967623459,
-12.9722599142832));
#71646=CARTESIAN_POINT('Ctrl Pts',(-17.7017145148158,-17.1035508497677,
-12.9738971246236));
#71647=CARTESIAN_POINT('Ctrl Pts',(-17.6365311652177,-17.1410205074514,
-12.9786448345478));
#71648=CARTESIAN_POINT('Ctrl Pts',(-17.5949591811586,-17.1668753695485,
-12.981802899346));
#71649=CARTESIAN_POINT('Ctrl Pts',(-17.4740684623494,-17.248003791619,-12.9913032927301));
#71650=CARTESIAN_POINT('Ctrl Pts',(-17.3975970787466,-17.3072940718698,
-12.9977324466284));
#71651=CARTESIAN_POINT('Ctrl Pts',(-17.2201704804253,-17.4654283083501,
-13.0133683538123));
#71652=CARTESIAN_POINT('Ctrl Pts',(-17.1245185358063,-17.5695536261855,
-13.0224360245941));
#71653=CARTESIAN_POINT('Ctrl Pts',(-17.0313564301591,-17.6938673115821,
-13.0319214934546));
#71654=CARTESIAN_POINT('Ctrl Pts',(-17.0229070028756,-17.7053830746888,
-13.0327890432953));
#71655=CARTESIAN_POINT('Ctrl Pts',(-17.009643570878,-17.7238488080858,-13.0341628067136));
#71656=CARTESIAN_POINT('Ctrl Pts',(-17.0047536494184,-17.7307434720371,
-13.0346719447464));
#71657=CARTESIAN_POINT('Ctrl Pts',(-16.9962016461544,-17.7429559287058,
-13.0355671802986));
#71658=CARTESIAN_POINT('Ctrl Pts',(-16.9925223775489,-17.7482614997871,
-13.0359539332874));
#71659=CARTESIAN_POINT('Ctrl Pts',(-16.9849620115875,-17.75927089851,-13.0367520292356));
#71660=CARTESIAN_POINT('Ctrl Pts',(-16.9810844044168,-17.7649770385774,
-13.0371632364698));
#71661=CARTESIAN_POINT('Ctrl Pts',(-16.9712013629442,-17.7796745876409,
-13.0382162124839));
#71662=CARTESIAN_POINT('Ctrl Pts',(-16.9652367467791,-17.7886933044593,
-13.0388564384312));
#71663=CARTESIAN_POINT('Ctrl Pts',(-16.9406197290176,-17.8265421970063,
-13.0415192153238));
#71664=CARTESIAN_POINT('Ctrl Pts',(-16.9226004333516,-17.8557792787245,
-13.0435181898367));
#71665=CARTESIAN_POINT('Ctrl Pts',(-16.8775013031238,-17.933105482106,-13.0486680993282));
#71666=CARTESIAN_POINT('Ctrl Pts',(-16.8515757658105,-17.9818386215875,
-13.0517795280847));
#71667=CARTESIAN_POINT('Ctrl Pts',(-16.7800131128559,-18.130054830611,-13.0609306890882));
#71668=CARTESIAN_POINT('Ctrl Pts',(-16.7401514618464,-18.2321198014625,
-13.0668217145879));
#71669=CARTESIAN_POINT('Ctrl Pts',(-16.6935607463832,-18.3855290571819,
-13.075550953093));
#71670=CARTESIAN_POINT('Ctrl Pts',(-16.6805271426218,-18.4347664445024,
-13.0783364533726));
#71671=CARTESIAN_POINT('Ctrl Pts',(-16.6658114747131,-18.4997477630116,
-13.082043323072));
#71672=CARTESIAN_POINT('Ctrl Pts',(-16.6625120047518,-18.5151094757731,
-13.082921877604));
#71673=CARTESIAN_POINT('Ctrl Pts',(-16.6488821168603,-18.5821965500195,
-13.0867737710449));
#71674=CARTESIAN_POINT('Ctrl Pts',(-16.6403167696737,-18.6342568320332,
-13.0898017226383));
#71675=CARTESIAN_POINT('Ctrl Pts',(-16.6326149766286,-18.695201364635,-13.093447320796));
#71676=CARTESIAN_POINT('Ctrl Pts',(-16.6315783129447,-18.7038315098328,
-13.0939659067662));
#71677=CARTESIAN_POINT('Ctrl Pts',(-16.6300882632132,-18.7169160805514,
-13.0947560408225));
#71678=CARTESIAN_POINT('Ctrl Pts',(-16.6295957989882,-18.7213660838256,
-13.0950254410843));
#71679=CARTESIAN_POINT('Ctrl Pts',(-16.6287367226327,-18.7293607579082,
-13.0955107063885));
#71680=CARTESIAN_POINT('Ctrl Pts',(-16.6283649412955,-18.7329048188489,
-13.0957262773786));
#71681=CARTESIAN_POINT('Ctrl Pts',(-16.6275760434057,-18.740612617913,-13.0961961048509));
#71682=CARTESIAN_POINT('Ctrl Pts',(-16.6271623284955,-18.7447766049649,
-13.0964505442747));
#71683=CARTESIAN_POINT('Ctrl Pts',(-16.6260337078267,-18.7564888772883,
-13.0971679225));
#71684=CARTESIAN_POINT('Ctrl Pts',(-16.6253470129127,-18.7640397273437,
-13.0976324004455));
#71685=CARTESIAN_POINT('Ctrl Pts',(-16.6214621617039,-18.8094612311245,
-13.1004377094568));
#71686=CARTESIAN_POINT('Ctrl Pts',(-16.6192439523349,-18.8474062032782,
-13.1028282950644));
#71687=CARTESIAN_POINT('Ctrl Pts',(-16.6152879487766,-18.973068866035,-13.1108564905582));
#71688=CARTESIAN_POINT('Ctrl Pts',(-16.6179805347711,-19.0608317096103,
-13.1166390871901));
#71689=CARTESIAN_POINT('Ctrl Pts',(-16.6422708687808,-19.3218393588444,
-13.1339594423221));
#71690=CARTESIAN_POINT('Ctrl Pts',(-16.6798383271981,-19.4928833380346,
-13.145406598618));
#71691=CARTESIAN_POINT('Ctrl Pts',(-16.7456646104199,-19.67914744913,-13.1575672761188));
#71692=CARTESIAN_POINT('Ctrl Pts',(-16.7537054664638,-19.7007687631953,
-13.158975435354));
#71693=CARTESIAN_POINT('Ctrl Pts',(-16.7655761013795,-19.7311583401141,
-13.1609504653947));
#71694=CARTESIAN_POINT('Ctrl Pts',(-16.7691141698648,-19.7400380973349,
-13.1615270559426));
#71695=CARTESIAN_POINT('Ctrl Pts',(-16.7749592022607,-19.7544236924032,
-13.1624604132948));
#71696=CARTESIAN_POINT('Ctrl Pts',(-16.7772294963945,-19.7599441977579,
-13.1628184123042));
#71697=CARTESIAN_POINT('Ctrl Pts',(-16.7820294182413,-19.77147690137,-13.1635659507681));
#71698=CARTESIAN_POINT('Ctrl Pts',(-16.7845635475733,-19.7774871672829,
-13.1639553328692));
#71699=CARTESIAN_POINT('Ctrl Pts',(-16.7906560133211,-19.7917523156977,
-13.1648790958912));
#71700=CARTESIAN_POINT('Ctrl Pts',(-16.7942392469403,-19.7999964781566,
-13.1654126227249));
#71701=CARTESIAN_POINT('Ctrl Pts',(-16.8064770449228,-19.8276692399912,
-13.1672025492852));
#71702=CARTESIAN_POINT('Ctrl Pts',(-16.8153720304585,-19.8469905715973,
-13.1684507132827));
#71703=CARTESIAN_POINT('Ctrl Pts',(-16.8912568177799,-20.0054915855231,
-13.1786847429151));
#71704=CARTESIAN_POINT('Ctrl Pts',(-16.9730038171536,-20.1370936072568,
-13.1871021016205));
#71705=CARTESIAN_POINT('Ctrl Pts',(-17.1527707598866,-20.3662522671283,
-13.2029188009421));
#71706=CARTESIAN_POINT('Ctrl Pts',(-17.2474062788223,-20.4654147187232,
-13.2103043431566));
#71707=CARTESIAN_POINT('Ctrl Pts',(-17.3627250384739,-20.564928057284,-13.2192364843212));
#71708=CARTESIAN_POINT('Ctrl Pts',(-17.3746370055784,-20.5749800231576,
-13.220158591548));
#71709=CARTESIAN_POINT('Ctrl Pts',(-17.3911125432161,-20.5885743563221,
-13.2214349466975));
#71710=CARTESIAN_POINT('Ctrl Pts',(-17.3955815638066,-20.592231213347,-13.2217812578595));
#71711=CARTESIAN_POINT('Ctrl Pts',(-17.4027117868424,-20.5980171044354,
-13.2223340458817));
#71712=CARTESIAN_POINT('Ctrl Pts',(-17.405363303654,-20.60015810629,-13.2225396671707));
#71713=CARTESIAN_POINT('Ctrl Pts',(-17.4108543852708,-20.6045700901351,
-13.2229656352164));
#71714=CARTESIAN_POINT('Ctrl Pts',(-17.4136946266629,-20.6068401557086,
-13.2231860471924));
#71715=CARTESIAN_POINT('Ctrl Pts',(-17.4204832407508,-20.6122373601705,
-13.2237130354384));
#71716=CARTESIAN_POINT('Ctrl Pts',(-17.4244369408101,-20.61535773715,-13.2240200893119));
#71717=CARTESIAN_POINT('Ctrl Pts',(-17.4378410712935,-20.6258592605778,
-13.2250614320295));
#71718=CARTESIAN_POINT('Ctrl Pts',(-17.447342866729,-20.6331740536974,-13.2258001867073));
#71719=CARTESIAN_POINT('Ctrl Pts',(-17.5586170524809,-20.7173406948873,
-13.2344532828878));
#71720=CARTESIAN_POINT('Ctrl Pts',(-17.6670612857956,-20.7849178593191,
-13.242886595689));
#71721=CARTESIAN_POINT('Ctrl Pts',(-17.9282980499113,-20.9166318025306,
-13.2622203688515));
#71722=CARTESIAN_POINT('Ctrl Pts',(-18.0838969379994,-20.9734646777314,
-13.2730158444569));
#71723=CARTESIAN_POINT('Ctrl Pts',(-18.2675087243459,-21.0170985742589,
-13.2846392240358));
#71724=CARTESIAN_POINT('Ctrl Pts',(-18.2905652612627,-21.0221719578198,
-13.286080842425));
#71725=CARTESIAN_POINT('Ctrl Pts',(-18.323158548674,-21.0287742742223,-13.2880942884745));
#71726=CARTESIAN_POINT('Ctrl Pts',(-18.3326276132522,-21.0306250975529,
-13.2886763525564));
#71727=CARTESIAN_POINT('Ctrl Pts',(-18.347991065657,-21.0335191393526,-13.2896161597697));
#71728=CARTESIAN_POINT('Ctrl Pts',(-18.3538777260398,-21.0346021902578,
-13.2899751688801));
#71729=CARTESIAN_POINT('Ctrl Pts',(-18.3661754505193,-21.0368108950247,
-13.2907229307289));
#71730=CARTESIAN_POINT('Ctrl Pts',(-18.3725872800356,-21.0379319774436,
-13.2911115343753));
#71731=CARTESIAN_POINT('Ctrl Pts',(-18.3877913579037,-21.0405181406197,
-13.292030061354));
#71732=CARTESIAN_POINT('Ctrl Pts',(-18.3965879341658,-21.041957307959,-13.2925591567417));
#71733=CARTESIAN_POINT('Ctrl Pts',(-18.4253810101607,-21.0464814836454,
-13.2942835669587));
#71734=CARTESIAN_POINT('Ctrl Pts',(-18.4454130618968,-21.0493354493858,
-13.2954715701017));
#71735=CARTESIAN_POINT('Ctrl Pts',(-18.4930790423714,-21.0554305453066,
-13.2982725966207));
#71736=CARTESIAN_POINT('Ctrl Pts',(-18.5207423175308,-21.0584150179696,
-13.2998776609134));
#71737=CARTESIAN_POINT('Ctrl Pts',(-18.7171650100066,-21.0756968227674,
-13.3111483189815));
#71738=CARTESIAN_POINT('Ctrl Pts',(-18.8870389590356,-21.0702429782238,
-13.3201754913812));
#71739=CARTESIAN_POINT('Ctrl Pts',(-19.1572101688511,-21.0288698788889,
-13.3351123390378));
#71740=CARTESIAN_POINT('Ctrl Pts',(-19.2586540326935,-21.0055889673471,
-13.3408766595485));
#71741=CARTESIAN_POINT('Ctrl Pts',(-19.3672203705736,-20.972102674751,-13.3476076668997));
#71742=CARTESIAN_POINT('Ctrl Pts',(-19.376457946993,-20.96918383707,-13.3481849790797));
#71743=CARTESIAN_POINT('Ctrl Pts',(-19.3900688505813,-20.964780164466,-13.3490428475197));
#71744=CARTESIAN_POINT('Ctrl Pts',(-19.394458024889,-20.9633442081365,-13.349320605287));
#71745=CARTESIAN_POINT('Ctrl Pts',(-19.4022370962683,-20.9607710093327,
-13.3498149256466));
#71746=CARTESIAN_POINT('Ctrl Pts',(-19.4056288476265,-20.9596395282995,
-13.3500311467298));
#71747=CARTESIAN_POINT('Ctrl Pts',(-19.4128905108622,-20.9571965913209,
-13.3504955737299));
#71748=CARTESIAN_POINT('Ctrl Pts',(-19.4167594388522,-20.9558825423636,
-13.3507439262314));
#71749=CARTESIAN_POINT('Ctrl Pts',(-19.4273710673343,-20.9522440926401,
-13.3514275598349));
#71750=CARTESIAN_POINT('Ctrl Pts',(-19.4341057912877,-20.9498968303757,
-13.3518641603594));
#71751=CARTESIAN_POINT('Ctrl Pts',(-19.4695225158455,-20.9373519286973,
-13.3541740836137));
#71752=CARTESIAN_POINT('Ctrl Pts',(-19.4979923761602,-20.9265711124939,
-13.3560791089139));
#71753=CARTESIAN_POINT('Ctrl Pts',(-19.6765789912471,-20.8545046253558,
-13.3682925365836));
#71754=CARTESIAN_POINT('Ctrl Pts',(-19.8194665385398,-20.7767576930581,
-13.3792085257959));
#71755=CARTESIAN_POINT('Ctrl Pts',(-20.0499070462781,-20.6146438519663,
-13.3976307853898));
#71756=CARTESIAN_POINT('Ctrl Pts',(-20.1417395844055,-20.5376460977423,
-13.4052584023651));
#71757=CARTESIAN_POINT('Ctrl Pts',(-20.2377288059876,-20.4422132330214,
-13.4135235941648));
#71758=CARTESIAN_POINT('Ctrl Pts',(-20.248746231174,-20.4310130756201,-13.414477400804));
#71759=CARTESIAN_POINT('Ctrl Pts',(-20.2652268079093,-20.413881815592,-13.4159123286463));
#71760=CARTESIAN_POINT('Ctrl Pts',(-20.2707822499913,-20.4080406240678,
-13.4163974664898));
#71761=CARTESIAN_POINT('Ctrl Pts',(-20.2806777374817,-20.3975164263434,
-13.4172642559059));
#71762=CARTESIAN_POINT('Ctrl Pts',(-20.285030193926,-20.3928452732211,-13.4176464401603));
#71763=CARTESIAN_POINT('Ctrl Pts',(-20.2942209517347,-20.3828916427895,
-13.418455499241));
#71764=CARTESIAN_POINT('Ctrl Pts',(-20.2990537165217,-20.3776041449064,
-13.4188821352738));
#71765=CARTESIAN_POINT('Ctrl Pts',(-20.3088371006349,-20.3667904970008,
-13.4197483457089));
#71766=CARTESIAN_POINT('Ctrl Pts',(-20.3137856956804,-20.3612626447143,
-13.4201878318702));
#71767=CARTESIAN_POINT('Ctrl Pts',(-20.3355743450282,-20.3366645339933,
-13.4221290260871));
#71768=CARTESIAN_POINT('Ctrl Pts',(-20.352099346437,-20.3173171212203,-13.4236176279517));
#71769=CARTESIAN_POINT('Ctrl Pts',(-20.4222713864287,-20.232095851272,-13.4300187482448));
#71770=CARTESIAN_POINT('Ctrl Pts',(-20.4722775149361,-20.1633212406356,
-13.4347859723443));
#71771=CARTESIAN_POINT('Ctrl Pts',(-20.5551898505232,-20.0335375724555,
-13.443273618919));
#71772=CARTESIAN_POINT('Ctrl Pts',(-20.5894925668684,-19.9735692243239,
-13.4470187497232));
#71773=CARTESIAN_POINT('Ctrl Pts',(-20.6594230944977,-19.8361307617998,
-13.4553933615768));
#71774=CARTESIAN_POINT('Ctrl Pts',(-20.6934048684955,-19.7580131654387,
-13.4600146201655));
#71775=CARTESIAN_POINT('Ctrl Pts',(-20.7225805467356,-19.6781104662135,
-13.4647889080502));
#71776=CARTESIAN_POINT('',(-20.8509991540683,-18.9538925310889,-12.4890563034253));
#71777=CARTESIAN_POINT('Ctrl Pts',(-20.7225805821191,-19.6781103693095,
-13.2445592932782));
#71778=CARTESIAN_POINT('Ctrl Pts',(-20.6962607934143,-19.7501917262988,
-13.2399327166672));
#71779=CARTESIAN_POINT('Ctrl Pts',(-20.6660544015046,-19.8207403796103,
-13.2353061400562));
#71780=CARTESIAN_POINT('Ctrl Pts',(-20.632174183212,-19.8893493319929,-13.2306795634452));
#71781=CARTESIAN_POINT('Ctrl Pts',(-20.6214444202636,-19.9110775802836,
-13.2292143405865));
#71782=CARTESIAN_POINT('Ctrl Pts',(-20.6103465168557,-19.9326114901367,
-13.2277491177279));
#71783=CARTESIAN_POINT('Ctrl Pts',(-20.5988881380091,-19.953938737006,-13.2262838948692));
#71784=CARTESIAN_POINT('Ctrl Pts',(-20.5645713376047,-20.017811897754,-13.2218956859383));
#71785=CARTESIAN_POINT('Ctrl Pts',(-20.526902233303,-20.0800446523181,-13.2175074770074));
#71786=CARTESIAN_POINT('Ctrl Pts',(-20.4860618340581,-20.1402627359456,
-13.2131192680765));
#71787=CARTESIAN_POINT('Ctrl Pts',(-20.4452820487372,-20.2003914459526,
-13.2087375719752));
#71788=CARTESIAN_POINT('Ctrl Pts',(-20.4013405804882,-20.2585110248676,
-13.2043558758739));
#71789=CARTESIAN_POINT('Ctrl Pts',(-20.3544642120277,-20.3142719029391,
-13.1999741797727));
#71790=CARTESIAN_POINT('Ctrl Pts',(-20.3076429270307,-20.3699672575413,
-13.195597632513));
#71791=CARTESIAN_POINT('Ctrl Pts',(-20.2578939016345,-20.4233090498181,
-13.1912210852534));
#71792=CARTESIAN_POINT('Ctrl Pts',(-20.2054860875596,-20.4739782173601,
-13.1868445379937));
#71793=CARTESIAN_POINT('Ctrl Pts',(-20.1531115097586,-20.5246152512524,
-13.1824707662767));
#71794=CARTESIAN_POINT('Ctrl Pts',(-20.0980818347927,-20.5725826889237,
-13.1780969945598));
#71795=CARTESIAN_POINT('Ctrl Pts',(-20.040704044844,-20.6175970518671,-13.1737232228428));
#71796=CARTESIAN_POINT('Ctrl Pts',(-19.9833437151495,-20.6625977167886,
-13.1693507820792));
#71797=CARTESIAN_POINT('Ctrl Pts',(-19.9236370683463,-20.7046467934755,
-13.1649783413157));
#71798=CARTESIAN_POINT('Ctrl Pts',(-19.8619241653156,-20.743501068182,-13.1606059005521));
#71799=CARTESIAN_POINT('Ctrl Pts',(-19.8002096842791,-20.7823563363966,
-13.1562333479848));
#71800=CARTESIAN_POINT('Ctrl Pts',(-19.7364892544385,-20.8180163851247,
-13.1518607954174));
#71801=CARTESIAN_POINT('Ctrl Pts',(-19.671130479885,-20.8502822402558,-13.1474882428501));
#71802=CARTESIAN_POINT('Ctrl Pts',(-19.60570387353,-20.8825815821084,-13.1431111522827));
#71803=CARTESIAN_POINT('Ctrl Pts',(-19.538635961093,-20.9114794832209,-13.1387340617154));
#71804=CARTESIAN_POINT('Ctrl Pts',(-19.4703166749595,-20.9368241116473,
-13.1343569711481));
#71805=CARTESIAN_POINT('Ctrl Pts',(-19.4019600771282,-20.9621825817159,
-13.1299774900891));
#71806=CARTESIAN_POINT('Ctrl Pts',(-19.3323512055625,-20.9839837711616,
-13.1255980090302));
#71807=CARTESIAN_POINT('Ctrl Pts',(-19.2618949953259,-21.0021258190438,
-13.1212185279712));
#71808=CARTESIAN_POINT('Ctrl Pts',(-19.1913139019297,-21.020300023584,-13.1168312843115));
#71809=CARTESIAN_POINT('Ctrl Pts',(-19.1198829437752,-21.0348020386143,
-13.1124440406518));
#71810=CARTESIAN_POINT('Ctrl Pts',(-19.048016498307,-21.0455812950041,-13.1080567969921));
#71811=CARTESIAN_POINT('Ctrl Pts',(-18.9991542404236,-21.0529101506624,
-13.1050738940573));
#71812=CARTESIAN_POINT('Ctrl Pts',(-18.9500908178362,-21.0585191746184,
-13.1020909911225));
#71813=CARTESIAN_POINT('Ctrl Pts',(-18.900956661124,-21.0624062341896,-13.0991080881877));
#71814=CARTESIAN_POINT('Ctrl Pts',(-18.8286744078926,-21.0681245662636,
-13.0947198792568));
#71815=CARTESIAN_POINT('Ctrl Pts',(-18.7559569381437,-21.0701362205188,
-13.0903316703259));
#71816=CARTESIAN_POINT('Ctrl Pts',(-18.6832169260197,-21.0683908144285,
-13.085943461395));
#71817=CARTESIAN_POINT('Ctrl Pts',(-18.6105848721342,-21.0666479988102,
-13.0815617652938));
#71818=CARTESIAN_POINT('Ctrl Pts',(-18.5379308205422,-21.0611592036425,
-13.0771800691925));
#71819=CARTESIAN_POINT('Ctrl Pts',(-18.4656714572673,-21.0519259018249,
-13.0727983730912));
#71820=CARTESIAN_POINT('Ctrl Pts',(-18.3934970044949,-21.0427034498716,
-13.0684218258316));
#71821=CARTESIAN_POINT('Ctrl Pts',(-18.3217167948298,-21.0297452929197,
-13.064045278572));
#71822=CARTESIAN_POINT('Ctrl Pts',(-18.2507446877307,-21.0131048743729,
-13.0596687313123));
#71823=CARTESIAN_POINT('Ctrl Pts',(-18.1798175901105,-20.9964750089376,
-13.0552949595953));
#71824=CARTESIAN_POINT('Ctrl Pts',(-18.1096980467018,-20.9761676251632,
-13.0509211878784));
#71825=CARTESIAN_POINT('Ctrl Pts',(-18.0407905817005,-20.9522874049448,
-13.0465474161614));
#71826=CARTESIAN_POINT('Ctrl Pts',(-17.9719040854722,-20.9284144515577,
-13.0421749753979));
#71827=CARTESIAN_POINT('Ctrl Pts',(-17.9042293909008,-20.9009709780647,
-13.0378025346343));
#71828=CARTESIAN_POINT('Ctrl Pts',(-17.8381550707622,-20.8701112748636,
-13.0334300938708));
#71829=CARTESIAN_POINT('Ctrl Pts',(-17.7720790610959,-20.8392507825765,
-13.0290575413034));
#71830=CARTESIAN_POINT('Ctrl Pts',(-17.7076039433215,-20.8049740930874,
-13.0246849887361));
#71831=CARTESIAN_POINT('Ctrl Pts',(-17.6450960002999,-20.7674826023504,
-13.0203124361687));
#71832=CARTESIAN_POINT('Ctrl Pts',(-17.5825231841773,-20.7299522015302,
-13.0159353456014));
#71833=CARTESIAN_POINT('Ctrl Pts',(-17.5219220335751,-20.6892005866782,
-13.0115582550341));
#71834=CARTESIAN_POINT('Ctrl Pts',(-17.4636312781366,-20.6454734454698,
-13.0071811644667));
#71835=CARTESIAN_POINT('Ctrl Pts',(-17.4053086879532,-20.6017224232466,
-13.0028016834078));
#71836=CARTESIAN_POINT('Ctrl Pts',(-17.3492993758005,-20.5549929484573,
-12.9984222023489));
#71837=CARTESIAN_POINT('Ctrl Pts',(-17.2959081742796,-20.5055703720129,
-12.9940427212899));
#71838=CARTESIAN_POINT('Ctrl Pts',(-17.2424223372125,-20.4560601943835,
-12.9896554776302));
#71839=CARTESIAN_POINT('Ctrl Pts',(-17.1915642147118,-20.4038477284533,
-12.9852682339705));
#71840=CARTESIAN_POINT('Ctrl Pts',(-17.1436006220654,-20.3492540279653,
-12.9808809903108));
#71841=CARTESIAN_POINT('Ctrl Pts',(-17.1109900008266,-20.3121355722699,
-12.9778980873759));
#71842=CARTESIAN_POINT('Ctrl Pts',(-17.0797165992413,-20.2739170566122,
-12.9749151844411));
#71843=CARTESIAN_POINT('Ctrl Pts',(-17.0498528101568,-20.2347069980877,
-12.9719322815063));
#71844=CARTESIAN_POINT('Ctrl Pts',(-17.0059195850955,-20.1770242867296,
-12.9675440725754));
#71845=CARTESIAN_POINT('Ctrl Pts',(-16.9648675150388,-20.1169692727541,
-12.9631558636445));
#71846=CARTESIAN_POINT('Ctrl Pts',(-16.926962336405,-20.0548616787018,-12.9587676547136));
#71847=CARTESIAN_POINT('Ctrl Pts',(-16.889113415341,-19.9928462626167,-12.9543859586124));
#71848=CARTESIAN_POINT('Ctrl Pts',(-16.8544023633226,-19.9287847222598,
-12.9500042625111));
#71849=CARTESIAN_POINT('Ctrl Pts',(-16.8230534861162,-19.8630282218873,
-12.9456225664098));
#71850=CARTESIAN_POINT('Ctrl Pts',(-16.7917414463352,-19.7973489906359,
-12.9412460191502));
#71851=CARTESIAN_POINT('Ctrl Pts',(-16.7637839395866,-19.7299791891848,
-12.9368694718905));
#71852=CARTESIAN_POINT('Ctrl Pts',(-16.739360042701,-19.661295735745,-12.9324929246309));
#71853=CARTESIAN_POINT('Ctrl Pts',(-16.7149516350957,-19.5926558403531,
-12.9281191529139));
#71854=CARTESIAN_POINT('Ctrl Pts',(-16.6940725522121,-19.5227043993277,
-12.9237453811969));
#71855=CARTESIAN_POINT('Ctrl Pts',(-16.6768537344171,-19.4518382158243,
-12.91937160948));
#71856=CARTESIAN_POINT('Ctrl Pts',(-16.6596401563663,-19.3809935971386,
-12.9149991687164));
#71857=CARTESIAN_POINT('Ctrl Pts',(-16.6460847459306,-19.3092352570616,
-12.9106267279528));
#71858=CARTESIAN_POINT('Ctrl Pts',(-16.6362680963764,-19.2369734382706,
-12.9062542871893));
#71859=CARTESIAN_POINT('Ctrl Pts',(-16.6264511958094,-19.164709771737,-12.9018817346219));
#71860=CARTESIAN_POINT('Ctrl Pts',(-16.620373308882,-19.0919430791857,-12.8975091820546));
#71861=CARTESIAN_POINT('Ctrl Pts',(-16.6180633554341,-19.0190903583474,
-12.8931366294872));
#71862=CARTESIAN_POINT('Ctrl Pts',(-16.6157510046294,-18.9461620282075,
-12.8887595389199));
#71863=CARTESIAN_POINT('Ctrl Pts',(-16.6172144102078,-18.8731479746871,
-12.8843824483526));
#71864=CARTESIAN_POINT('Ctrl Pts',(-16.6224303356468,-18.8004660018901,
-12.8800053577853));
#71865=CARTESIAN_POINT('Ctrl Pts',(-16.6276491096962,-18.7277443347702,
-12.8756258767263));
#71866=CARTESIAN_POINT('Ctrl Pts',(-16.6366244245267,-18.6553555885067,
-12.8712463956674));
#71867=CARTESIAN_POINT('Ctrl Pts',(-16.6492813452851,-18.5837105341124,
-12.8668669146084));
#71868=CARTESIAN_POINT('Ctrl Pts',(-16.6619607003506,-18.5119384893401,
-12.8624796709487));
#71869=CARTESIAN_POINT('Ctrl Pts',(-16.6783345842871,-18.4409132392692,
-12.858092427289));
#71870=CARTESIAN_POINT('Ctrl Pts',(-16.6982774637591,-18.3710329136339,
-12.8537051836292));
#71871=CARTESIAN_POINT('Ctrl Pts',(-16.7118367001087,-18.3235210258541,
-12.8507222806944));
#71872=CARTESIAN_POINT('Ctrl Pts',(-16.7270447244344,-18.27653808659,-12.8477393777596));
#71873=CARTESIAN_POINT('Ctrl Pts',(-16.7438494759073,-18.2302037050153,
-12.8447564748248));
#71874=CARTESIAN_POINT('Ctrl Pts',(-16.7685712862064,-18.1620402577033,
-12.8403682658939));
#71875=CARTESIAN_POINT('Ctrl Pts',(-16.7968473421401,-18.0950153233851,
-12.835980056963));
#71876=CARTESIAN_POINT('Ctrl Pts',(-16.8285526457323,-18.0295254040819,
-12.8315918480321));
#71877=CARTESIAN_POINT('Ctrl Pts',(-16.8602108933972,-17.9641326826773,
-12.8272101519309));
#71878=CARTESIAN_POINT('Ctrl Pts',(-16.8952880767684,-17.9002708843009,
-12.8228284558296));
#71879=CARTESIAN_POINT('Ctrl Pts',(-16.9336103347364,-17.8383186931567,
-12.8184467597283));
#71880=CARTESIAN_POINT('Ctrl Pts',(-16.9718875610016,-17.7764393007675,
-12.8140702124687));
#71881=CARTESIAN_POINT('Ctrl Pts',(-17.0134020343727,-17.7164654662072,
-12.8096936652091));
#71882=CARTESIAN_POINT('Ctrl Pts',(-17.057933757175,-17.6587517834296,-12.8053171179494));
#71883=CARTESIAN_POINT('Ctrl Pts',(-17.1024372386059,-17.6010747018308,
-12.8009433462325));
#71884=CARTESIAN_POINT('Ctrl Pts',(-17.149953878891,-17.5456553090191,-12.7965695745155));
#71885=CARTESIAN_POINT('Ctrl Pts',(-17.2002209049089,-17.4928184871437,
-12.7921958027985));
#71886=CARTESIAN_POINT('Ctrl Pts',(-17.250472634502,-17.4399977436907,-12.787823362035));
#71887=CARTESIAN_POINT('Ctrl Pts',(-17.3034727559331,-17.3897583602254,
-12.7834509212714));
#71888=CARTESIAN_POINT('Ctrl Pts',(-17.3589199436392,-17.3423901595111,
-12.7790784805079));
#71889=CARTESIAN_POINT('Ctrl Pts',(-17.4143685491361,-17.2950207475866,
-12.7747059279405));
#71890=CARTESIAN_POINT('Ctrl Pts',(-17.4722639770754,-17.2505229759786,
-12.7703333753732));
#71891=CARTESIAN_POINT('Ctrl Pts',(-17.5322712521177,-17.2091468746583,
-12.7659608228059));
#71892=CARTESIAN_POINT('Ctrl Pts',(-17.5923408049735,-17.1677278316595,
-12.7615837322385));
#71893=CARTESIAN_POINT('Ctrl Pts',(-17.6545261829435,-17.1294372018124,
-12.7572066416712));
#71894=CARTESIAN_POINT('Ctrl Pts',(-17.7184635014064,-17.0944815963161,
-12.7528295511039));
#71895=CARTESIAN_POINT('Ctrl Pts',(-17.782435738412,-17.0595069002663,-12.7484500700449));
#71896=CARTESIAN_POINT('Ctrl Pts',(-17.8481613859395,-17.0278710642731,
-12.744070588986));
#71897=CARTESIAN_POINT('Ctrl Pts',(-17.9152544897584,-16.9997334225421,
-12.7396911079271));
#71898=CARTESIAN_POINT('Ctrl Pts',(-17.9824665156535,-16.97154590703,-12.7353038642674));
#71899=CARTESIAN_POINT('Ctrl Pts',(-18.0510503837931,-16.9468691314342,
-12.7309166206076));
#71900=CARTESIAN_POINT('Ctrl Pts',(-18.1206033812626,-16.9258130421598,
-12.7265293769479));
#71901=CARTESIAN_POINT('Ctrl Pts',(-18.1678927174312,-16.9114969304131,
-12.7235464740131));
#71902=CARTESIAN_POINT('Ctrl Pts',(-18.2156297492658,-16.8988534982272,
-12.7205635710783));
#71903=CARTESIAN_POINT('Ctrl Pts',(-18.2636857248404,-16.887903712861,-12.7175806681434));
#71904=CARTESIAN_POINT('Ctrl Pts',(-18.3343818439591,-16.8717952618032,
-12.7131924592126));
#71905=CARTESIAN_POINT('Ctrl Pts',(-18.4060444995739,-16.8592916243426,
-12.7088042502817));
#71906=CARTESIAN_POINT('Ctrl Pts',(-18.4782726371994,-16.8505023159863,
-12.7044160413508));
#71907=CARTESIAN_POINT('Ctrl Pts',(-18.5503935762929,-16.8417260524208,
-12.7000343452495));
#71908=CARTESIAN_POINT('Ctrl Pts',(-18.623077856446,-16.8366532323251,-12.6956526491482));
#71909=CARTESIAN_POINT('Ctrl Pts',(-18.6959129564504,-16.8353426405973,
-12.691270953047));
#71910=CARTESIAN_POINT('Ctrl Pts',(-18.768662469416,-16.8340335889191,-12.6868944057873));
#71911=CARTESIAN_POINT('Ctrl Pts',(-18.8415619702677,-16.8364779920626,
-12.6825178585277));
#71912=CARTESIAN_POINT('Ctrl Pts',(-18.9141942210373,-16.8426828017805,
-12.6781413112681));
#71913=CARTESIAN_POINT('Ctrl Pts',(-18.9867804094891,-16.8488836764982,
-12.6737675395511));
#71914=CARTESIAN_POINT('Ctrl Pts',(-19.0590992046967,-16.8588401850895,
-12.6693937678341));
#71915=CARTESIAN_POINT('Ctrl Pts',(-19.1307351980795,-16.8725072294896,
-12.6650199961172));
#71916=CARTESIAN_POINT('Ctrl Pts',(-19.202349392389,-16.8861701149623,-12.6606475553536));
#71917=CARTESIAN_POINT('Ctrl Pts',(-19.2732807238323,-16.9035412042303,
-12.6562751145901));
#71918=CARTESIAN_POINT('Ctrl Pts',(-19.3431223955191,-16.9245240057458,
-12.6519026738265));
#71919=CARTESIAN_POINT('Ctrl Pts',(-19.4129658530651,-16.9455073437939,
-12.6475301212592));
#71920=CARTESIAN_POINT('Ctrl Pts',(-19.4817191341323,-16.9701024367362,
-12.6431575686918));
#71921=CARTESIAN_POINT('Ctrl Pts',(-19.5489906872852,-16.9981629598049,
-12.6387850161245));
#71922=CARTESIAN_POINT('Ctrl Pts',(-19.6163320573932,-17.0262526051427,
-12.6344079255571));
#71923=CARTESIAN_POINT('Ctrl Pts',(-19.6821881831272,-17.0578146752691,
-12.6300308349898));
#71924=CARTESIAN_POINT('Ctrl Pts',(-19.746188373322,-17.0926550355268,-12.6256537444225));
#71925=CARTESIAN_POINT('Ctrl Pts',(-19.8102235163959,-17.1275144233983,
-12.6212742633636));
#71926=CARTESIAN_POINT('Ctrl Pts',(-19.8724002944077,-17.1656554136576,
-12.6168947823046));
#71927=CARTESIAN_POINT('Ctrl Pts',(-19.932375822801,-17.2068397244591,-12.6125153012457));
#71928=CARTESIAN_POINT('Ctrl Pts',(-19.9924576574157,-17.248097034175,-12.608128057586));
#71929=CARTESIAN_POINT('Ctrl Pts',(-20.0503300675354,-17.29240814305,-12.6037408139262));
#71930=CARTESIAN_POINT('Ctrl Pts',(-20.1056826247701,-17.3394939451575,
-12.5993535702665));
#71931=CARTESIAN_POINT('Ctrl Pts',(-20.1433170299302,-17.3715077534137,
-12.5963706673317));
#71932=CARTESIAN_POINT('Ctrl Pts',(-20.1797873054597,-17.4048033925969,
-12.5933877643969));
#71933=CARTESIAN_POINT('Ctrl Pts',(-20.2150061302366,-17.4392839518926,
-12.590404861462));
#71934=CARTESIAN_POINT('Ctrl Pts',(-20.2660558507877,-17.4892635559152,
-12.5860811407752));
#71935=CARTESIAN_POINT('Ctrl Pts',(-20.3146860821101,-17.5419415318573,
-12.5817574200883));
#71936=CARTESIAN_POINT('Ctrl Pts',(-20.3605919747976,-17.5970507214202,
-12.5774336994015));
#71937=CARTESIAN_POINT('Ctrl Pts',(-20.4064369112149,-17.652086734089,-12.5731157199795));
#71938=CARTESIAN_POINT('Ctrl Pts',(-20.4495643625502,-17.7095471849218,
-12.5687977405574));
#71939=CARTESIAN_POINT('Ctrl Pts',(-20.4897052944034,-17.7691272599286,
-12.5644797611354));
#71940=CARTESIAN_POINT('Ctrl Pts',(-20.5298070691322,-17.8286492150986,
-12.5601659938641));
#71941=CARTESIAN_POINT('Ctrl Pts',(-20.5669278234433,-17.8902862851976,
-12.5558522265929));
#71942=CARTESIAN_POINT('Ctrl Pts',(-20.6008391323988,-17.9537011200325,
-12.5515384593216));
#71943=CARTESIAN_POINT('Ctrl Pts',(-20.6347293023105,-18.0170764244271,
-12.5472273810918));
#71944=CARTESIAN_POINT('Ctrl Pts',(-20.6654137615195,-18.0822268576,-12.542916302862));
#71945=CARTESIAN_POINT('Ctrl Pts',(-20.6927087374024,-18.1487882707383,
-12.5386052246321));
#71946=CARTESIAN_POINT('Ctrl Pts',(-20.720007692024,-18.2153593864121,-12.5342935179843));
#71947=CARTESIAN_POINT('Ctrl Pts',(-20.7439159714601,-18.2833414390349,
-12.5299818113365));
#71948=CARTESIAN_POINT('Ctrl Pts',(-20.7642975065945,-18.3523492393767,
-12.5256701046887));
#71949=CARTESIAN_POINT('Ctrl Pts',(-20.7846795217661,-18.4213586650285,
-12.5213582964892));
#71950=CARTESIAN_POINT('Ctrl Pts',(-20.8015344966334,-18.4913934058167,
-12.5170464882897));
#71951=CARTESIAN_POINT('Ctrl Pts',(-20.8147766394152,-18.5620543924287,
-12.5127346800901));
#71952=CARTESIAN_POINT('Ctrl Pts',(-20.828033543779,-18.6327941478605,-12.5084180653339));
#71953=CARTESIAN_POINT('Ctrl Pts',(-20.8376694934189,-18.7041610510436,
-12.5041014505776));
#71954=CARTESIAN_POINT('Ctrl Pts',(-20.8436502754155,-18.7757481477,-12.4997848358213));
#71955=CARTESIAN_POINT('Ctrl Pts',(-20.8486051622908,-18.8350557709941,
-12.496208658356));
#71956=CARTESIAN_POINT('Ctrl Pts',(-20.8510522363742,-18.8945142745419,
-12.4926324808906));
#71957=CARTESIAN_POINT('Ctrl Pts',(-20.8509991540683,-18.9538925310889,
-12.4890563034253));
#71958=CARTESIAN_POINT('Ctrl Pts',(-20.8516473850063,-18.9538935158916,
-12.4890562790225));
#71959=CARTESIAN_POINT('Ctrl Pts',(-20.8529700926033,-19.0968822287437,
-12.4804472042752));
#71960=CARTESIAN_POINT('Ctrl Pts',(-20.8300641645468,-19.3437931350663,
-12.4655558047043));
#71961=CARTESIAN_POINT('Ctrl Pts',(-20.7608946003787,-19.5811887556435,
-12.4506644051334));
#71962=CARTESIAN_POINT('Ctrl Pts',(-20.7242504220745,-19.678735851896,-12.4443820803097));
#71963=CARTESIAN_POINT('Origin',(-18.734,-18.952,0.));
#71964=CARTESIAN_POINT('',(-20.7225805826898,-19.6781103677465,-11.642549326843));
#71965=CARTESIAN_POINT('',(-20.7225805820713,-19.6781103694405,-11.8674650853572));
#71966=CARTESIAN_POINT('',(-20.7225805821191,-19.6781103693095,0.));
#71967=CARTESIAN_POINT('',(-20.8509993992253,-18.9504051082612,-11.9120635502395));
#71968=CARTESIAN_POINT('Ctrl Pts',(-20.7225805820713,-19.6781103694405,
-11.8674650853572));
#71969=CARTESIAN_POINT('Ctrl Pts',(-20.7358715470792,-19.6417107309776,
-11.8699797732346));
#71970=CARTESIAN_POINT('Ctrl Pts',(-20.7481612630639,-19.604951226548,-11.8724727008059));
#71971=CARTESIAN_POINT('Ctrl Pts',(-20.7623062774745,-19.5584322024437,
-11.8755658152096));
#71972=CARTESIAN_POINT('Ctrl Pts',(-20.7651109560046,-19.5489712391965,
-11.8761917407254));
#71973=CARTESIAN_POINT('Ctrl Pts',(-20.783378893993,-19.4857290083341,-11.8803546635274));
#71974=CARTESIAN_POINT('Ctrl Pts',(-20.7967716263503,-19.4313690076842,
-11.8838304877392));
#71975=CARTESIAN_POINT('Ctrl Pts',(-20.8104073115161,-19.3647545756929,
-11.887969560528));
#71976=CARTESIAN_POINT('Ctrl Pts',(-20.8127188708028,-19.3529507807812,
-11.8886984932715));
#71977=CARTESIAN_POINT('Ctrl Pts',(-20.8163752184754,-19.3333978114117,
-11.8898986987927));
#71978=CARTESIAN_POINT('Ctrl Pts',(-20.8177776237672,-19.3256598163581,
-11.8903717987834));
#71979=CARTESIAN_POINT('Ctrl Pts',(-20.8202374523177,-19.3116426489251,
-11.8912254707796));
#71980=CARTESIAN_POINT('Ctrl Pts',(-20.8213097198868,-19.3053662080856,
-11.8916065107796));
#71981=CARTESIAN_POINT('Ctrl Pts',(-20.8233364632863,-19.2931716236168,
-11.8923445323753));
#71982=CARTESIAN_POINT('Ctrl Pts',(-20.8242941503961,-19.2872540820544,
-11.892701612527));
#71983=CARTESIAN_POINT('Ctrl Pts',(-20.8263396796084,-19.2742651871561,
-11.8934831274235));
#71984=CARTESIAN_POINT('Ctrl Pts',(-20.827416838552,-19.2671922075359,-11.8939072211355));
#71985=CARTESIAN_POINT('Ctrl Pts',(-20.8299772097504,-19.2497876328722,
-11.894947251902));
#71986=CARTESIAN_POINT('Ctrl Pts',(-20.8314199210973,-19.2394502017417,
-11.8955619130377));
#71987=CARTESIAN_POINT('Ctrl Pts',(-20.8449846075371,-19.1367106455658,
-11.9016414582525));
#71988=CARTESIAN_POINT('Ctrl Pts',(-20.8510696177588,-19.0436105526441,
-11.9069088192729));
#71989=CARTESIAN_POINT('Ctrl Pts',(-20.8509993992253,-18.9504051082612,
-11.9120635502395));
#71990=CARTESIAN_POINT('Ctrl Pts',(-20.8509994011072,-18.9504076081963,
-11.9120634119805));
#71991=CARTESIAN_POINT('Ctrl Pts',(-20.8509185676265,-18.8429438358049,
-11.9180067026759));
#71992=CARTESIAN_POINT('Ctrl Pts',(-20.8426553590784,-18.7356392271031,
-11.9237827343211));
#71993=CARTESIAN_POINT('Ctrl Pts',(-20.8144662881294,-18.5528019122291,
-11.9338768813632));
#71994=CARTESIAN_POINT('Ctrl Pts',(-20.7984544823587,-18.476894838746,-11.9381478592865));
#71995=CARTESIAN_POINT('Ctrl Pts',(-20.7691437057061,-18.3679398005603,
-11.9446066414929));
#71996=CARTESIAN_POINT('Ctrl Pts',(-20.7591179340521,-18.334073432349,-11.9466619632899));
#71997=CARTESIAN_POINT('Ctrl Pts',(-20.7459662609387,-18.2934137430804,
-11.9492053394917));
#71998=CARTESIAN_POINT('Ctrl Pts',(-20.7436448499687,-18.2863637132412,
-11.9496491277717));
#71999=CARTESIAN_POINT('Ctrl Pts',(-20.7399678682761,-18.2753914484512,
-11.9503443826599));
#72000=CARTESIAN_POINT('Ctrl Pts',(-20.7386377313515,-18.2714606653927,
-11.950594373282));
#72001=CARTESIAN_POINT('Ctrl Pts',(-20.7361428095416,-18.2641585262246,
-11.9510605279638));
#72002=CARTESIAN_POINT('Ctrl Pts',(-20.7349810585352,-18.2607861939944,
-11.9512765119146));
#72003=CARTESIAN_POINT('Ctrl Pts',(-20.7323265932119,-18.2531435839721,
-11.9517675738904));
#72004=CARTESIAN_POINT('Ctrl Pts',(-20.7308287180436,-18.2488751652235,
-11.9520429539471));
#72005=CARTESIAN_POINT('Ctrl Pts',(-20.7263403321082,-18.2362148587465,
-11.9528630037925));
#72006=CARTESIAN_POINT('Ctrl Pts',(-20.723310560138,-18.2278371341262,-11.9534099211958));
#72007=CARTESIAN_POINT('Ctrl Pts',(-20.70003653577,-18.1647297046504,-11.9575606454482));
#72008=CARTESIAN_POINT('Ctrl Pts',(-20.6775917875363,-18.1108437544836,
-11.9612804744289));
#72009=CARTESIAN_POINT('Ctrl Pts',(-20.6438613574187,-18.0384453847687,
-11.966458491192));
#72010=CARTESIAN_POINT('Ctrl Pts',(-20.6344729737546,-18.0190718803266,
-11.9678624389679));
#72011=CARTESIAN_POINT('Ctrl Pts',(-20.5649713374984,-17.8810553648092,
-11.9779817419938));
#72012=CARTESIAN_POINT('Ctrl Pts',(-20.4940849116522,-17.7681574140124,
-11.9868646309309));
#72013=CARTESIAN_POINT('Ctrl Pts',(-20.3732623415019,-17.6108137189589,
-11.9997138529784));
#72014=CARTESIAN_POINT('Ctrl Pts',(-20.3310694303964,-17.5608378175314,
-12.0038810957337));
#72015=CARTESIAN_POINT('Ctrl Pts',(-20.2691983534546,-17.4940862824816,
-12.0095592717183));
#72016=CARTESIAN_POINT('Ctrl Pts',(-20.2514281028702,-17.4755995006899,
-12.0111449690918));
#72017=CARTESIAN_POINT('Ctrl Pts',(-20.2199337027648,-17.4440046845269,
-12.0138788298085));
#72018=CARTESIAN_POINT('Ctrl Pts',(-20.2063613374684,-17.4307501950048,
-12.0150333647132));
#72019=CARTESIAN_POINT('Ctrl Pts',(-20.1863980443352,-17.4117719526879,
-12.0166981609527));
#72020=CARTESIAN_POINT('Ctrl Pts',(-20.1801478896024,-17.4059020724114,
-12.0172147447383));
#72021=CARTESIAN_POINT('Ctrl Pts',(-20.1691113632873,-17.3956625130229,
-12.0181189044961));
#72022=CARTESIAN_POINT('Ctrl Pts',(-20.1643402989295,-17.3912765686663,
-12.0185071748868));
#72023=CARTESIAN_POINT('Ctrl Pts',(-20.1550953315577,-17.3828558537133,
-12.0192545811365));
#72024=CARTESIAN_POINT('Ctrl Pts',(-20.1506242038972,-17.3788181416987,
-12.0196138398409));
#72025=CARTESIAN_POINT('Ctrl Pts',(-20.1387915016344,-17.3682238110123,
-12.0205588518216));
#72026=CARTESIAN_POINT('Ctrl Pts',(-20.1314012045182,-17.3616993811009,
-12.0211432503674));
#72027=CARTESIAN_POINT('Ctrl Pts',(-20.1052286970545,-17.3389166334173,
-12.0231927943456));
#72028=CARTESIAN_POINT('Ctrl Pts',(-20.0862057148745,-17.3229371196022,
-12.0246464249312));
#72029=CARTESIAN_POINT('Ctrl Pts',(-19.9417783239518,-17.2058899267861,
-12.0354289966536));
#72030=CARTESIAN_POINT('Ctrl Pts',(-19.8054879199467,-17.1190926754184,
-12.0441454916573));
#72031=CARTESIAN_POINT('Ctrl Pts',(-19.543790477347,-16.9916877723254,-12.0599582577842));
#72032=CARTESIAN_POINT('Ctrl Pts',(-19.4219457147379,-16.9456835890036,
-12.0670290975834));
#72033=CARTESIAN_POINT('Ctrl Pts',(-19.2852115225785,-16.9079852652148,
-12.0753993043172));
#72034=CARTESIAN_POINT('Ctrl Pts',(-19.2737227985241,-16.904921675954,-12.0761059186987));
#72035=CARTESIAN_POINT('Ctrl Pts',(-19.2573483935927,-16.9007026898369,
-12.077118546535));
#72036=CARTESIAN_POINT('Ctrl Pts',(-19.252483228653,-16.8994675797488,-12.0774201088643));
#72037=CARTESIAN_POINT('Ctrl Pts',(-19.2440893407327,-16.8973683875234,
-12.0779416567103));
#72038=CARTESIAN_POINT('Ctrl Pts',(-19.2405626645072,-16.8964960556362,
-12.0781611676606));
#72039=CARTESIAN_POINT('Ctrl Pts',(-19.2337187710189,-16.8948218850486,
-12.0785879224804));
#72040=CARTESIAN_POINT('Ctrl Pts',(-19.2304018533018,-16.8940189878427,
-12.0787950981116));
#72041=CARTESIAN_POINT('Ctrl Pts',(-19.221443932642,-16.8918735388113,-12.0793555220617));
#72042=CARTESIAN_POINT('Ctrl Pts',(-19.2157993800231,-16.8905461491583,
-12.0797096280388));
#72043=CARTESIAN_POINT('Ctrl Pts',(-19.1948080548063,-16.8857006901206,
-12.0810299257304));
#72044=CARTESIAN_POINT('Ctrl Pts',(-19.1794280713751,-16.8823307749749,
-12.0820040751469));
#72045=CARTESIAN_POINT('Ctrl Pts',(-19.0338793528071,-16.8521369622244,
-12.091277707838));
#72046=CARTESIAN_POINT('Ctrl Pts',(-18.9015049597613,-16.8374578893284,
-12.1001050363254));
#72047=CARTESIAN_POINT('Ctrl Pts',(-18.6105816054926,-16.8326966396408,
-12.1193232908383));
#72048=CARTESIAN_POINT('Ctrl Pts',(-18.4527006870236,-16.8478214602303,
-12.1296096473111));
#72049=CARTESIAN_POINT('Ctrl Pts',(-18.2771319967909,-16.8847764096748,
-12.1406290920443));
#72050=CARTESIAN_POINT('Ctrl Pts',(-18.2563771364257,-16.889472861555,-12.1419259562897));
#72051=CARTESIAN_POINT('Ctrl Pts',(-18.2269580599202,-16.8965977763712,
-12.1437565121233));
#72052=CARTESIAN_POINT('Ctrl Pts',(-18.2182335895534,-16.8987696564558,
-12.1442984128683));
#72053=CARTESIAN_POINT('Ctrl Pts',(-18.2032036125933,-16.9026130812662,
-12.1452303719699));
#72054=CARTESIAN_POINT('Ctrl Pts',(-18.196891560507,-16.904258299183,-12.1456212745695));
#72055=CARTESIAN_POINT('Ctrl Pts',(-18.1848184377886,-16.9074647869958,
-12.1463680607121));
#72056=CARTESIAN_POINT('Ctrl Pts',(-18.179056178119,-16.9090212969375,-12.1467240941382));
#72057=CARTESIAN_POINT('Ctrl Pts',(-18.1640851621782,-16.9131333031989,
-12.1476481293907));
#72058=CARTESIAN_POINT('Ctrl Pts',(-18.1548869244608,-16.9157268405281,
-12.1482148913496));
#72059=CARTESIAN_POINT('Ctrl Pts',(-18.1235594148199,-16.9247893967345,
-12.1501421194037));
#72060=CARTESIAN_POINT('Ctrl Pts',(-18.1015179135435,-16.9315577192699,
-12.151492835393));
#72061=CARTESIAN_POINT('Ctrl Pts',(-17.9135613355801,-16.9926512524357,
-12.1629764456236));
#72062=CARTESIAN_POINT('Ctrl Pts',(-17.7548460951913,-17.0669452295633,
-12.1723674309809));
#72063=CARTESIAN_POINT('Ctrl Pts',(-17.5328552153039,-17.206542941225,-12.1866338937454));
#72064=CARTESIAN_POINT('Ctrl Pts',(-17.4616422455476,-17.2577531318441,
-12.1914296539073));
#72065=CARTESIAN_POINT('Ctrl Pts',(-17.3644107249343,-17.3372687796213,
-12.1985998549312));
#72066=CARTESIAN_POINT('Ctrl Pts',(-17.3356625658025,-17.362099464542,-12.2008059067099));
#72067=CARTESIAN_POINT('Ctrl Pts',(-17.3019982132014,-17.3927959238269,
-12.2035164515418));
#72068=CARTESIAN_POINT('Ctrl Pts',(-17.2964241144743,-17.3979337086322,
-12.2039695904049));
#72069=CARTESIAN_POINT('Ctrl Pts',(-17.287816433903,-17.40595355793,-12.2046763184344));
#72070=CARTESIAN_POINT('Ctrl Pts',(-17.2847635348026,-17.4088149251846,
-12.2049283515191));
#72071=CARTESIAN_POINT('Ctrl Pts',(-17.2791263015234,-17.4141299726935,
-12.2053963366021));
#72072=CARTESIAN_POINT('Ctrl Pts',(-17.2765396723192,-17.416581134653,-12.2056120960131));
#72073=CARTESIAN_POINT('Ctrl Pts',(-17.2707169491088,-17.4221268805651,
-12.2061001047623));
#72074=CARTESIAN_POINT('Ctrl Pts',(-17.2674844956563,-17.4252251890792,
-12.206372640274));
#72075=CARTESIAN_POINT('Ctrl Pts',(-17.2580046488534,-17.4343695087406,
-12.2071766206417));
#72076=CARTESIAN_POINT('Ctrl Pts',(-17.2517847304922,-17.4404436915919,
-12.2077101870163));
#72077=CARTESIAN_POINT('Ctrl Pts',(-17.2080430168751,-17.483690103548,-12.2115044535058));
#72078=CARTESIAN_POINT('Ctrl Pts',(-17.1718896218182,-17.5222137140302,
-12.2148603229745));
#72079=CARTESIAN_POINT('Ctrl Pts',(-17.1270154340751,-17.5737652377432,
-12.2192759565411));
#72080=CARTESIAN_POINT('Ctrl Pts',(-17.1169426633622,-17.5855974209795,
-12.2202846082135));
#72081=CARTESIAN_POINT('Ctrl Pts',(-17.0206797985266,-17.7012298272086,
-12.2300877104767));
#72082=CARTESIAN_POINT('Ctrl Pts',(-16.9444672921623,-17.8129357490622,
-12.2391142900666));
#72083=CARTESIAN_POINT('Ctrl Pts',(-16.8324364319377,-18.0164623445212,
-12.254226853012));
#72084=CARTESIAN_POINT('Ctrl Pts',(-16.7914098361147,-18.1049328999886,
-12.2604206720449));
#72085=CARTESIAN_POINT('Ctrl Pts',(-16.7488927238891,-18.2161291225741,
-12.2677349921378));
#72086=CARTESIAN_POINT('Ctrl Pts',(-16.7414776561936,-18.2364501346267,
-12.2690536179719));
#72087=CARTESIAN_POINT('Ctrl Pts',(-16.7314035750793,-18.2654299315242,
-12.270909249224));
#72088=CARTESIAN_POINT('Ctrl Pts',(-16.7284868551709,-18.2739971018309,
-12.2714547729041));
#72089=CARTESIAN_POINT('Ctrl Pts',(-16.7235591097719,-18.2887812458655,
-12.2723910073258));
#72090=CARTESIAN_POINT('Ctrl Pts',(-16.721521782423,-18.294989258687,-12.2727825828778));
#72091=CARTESIAN_POINT('Ctrl Pts',(-16.7176820909712,-18.306874763982,-12.2735293320088));
#72092=CARTESIAN_POINT('Ctrl Pts',(-16.7158748880513,-18.3125506165016,
-12.2738846618351));
#72093=CARTESIAN_POINT('Ctrl Pts',(-16.7112508296161,-18.3272881934851,
-12.2748040273872));
#72094=CARTESIAN_POINT('Ctrl Pts',(-16.7084708834987,-18.336361428961,-12.2753668484514));
#72095=CARTESIAN_POINT('Ctrl Pts',(-16.6992635842597,-18.3671499602183,
-12.2772661542599));
#72096=CARTESIAN_POINT('Ctrl Pts',(-16.6931235535876,-18.3889500560984,
-12.2785932742696));
#72097=CARTESIAN_POINT('Ctrl Pts',(-16.6413731965901,-18.5846716186548,
-12.2903612435084));
#72098=CARTESIAN_POINT('Ctrl Pts',(-16.6177427928168,-18.7636413725187,
-12.3000071994611));
#72099=CARTESIAN_POINT('Ctrl Pts',(-16.6166782209977,-19.0274760084611,
-12.3143734482994));
#72100=CARTESIAN_POINT('Ctrl Pts',(-16.6213412674197,-19.1114333725433,
-12.3189820059042));
#72101=CARTESIAN_POINT('Ctrl Pts',(-16.6352307957032,-19.231696336893,-12.3258994678031));
#72102=CARTESIAN_POINT('Ctrl Pts',(-16.6404478918399,-19.2683880641553,
-12.3280532474319));
#72103=CARTESIAN_POINT('Ctrl Pts',(-16.6478796142739,-19.3123434444918,
-12.3307058467947));
#72104=CARTESIAN_POINT('Ctrl Pts',(-16.6491740493474,-19.3197586346467,
-12.3311558322912));
#72105=CARTESIAN_POINT('Ctrl Pts',(-16.6512474400778,-19.3312732327306,
-12.3318586922956));
#72106=CARTESIAN_POINT('Ctrl Pts',(-16.6519990317559,-19.3353775925498,
-12.3321100379411));
#72107=CARTESIAN_POINT('Ctrl Pts',(-16.6534151877111,-19.3429840731354,
-12.3325774007549));
#72108=CARTESIAN_POINT('Ctrl Pts',(-16.6540764648268,-19.3464867473232,
-12.3327932295165));
#72109=CARTESIAN_POINT('Ctrl Pts',(-16.6555911984728,-19.3544003457163,
-12.3332822376755));
#72110=CARTESIAN_POINT('Ctrl Pts',(-16.6564498471733,-19.3588102089762,
-12.3335557084669));
#72111=CARTESIAN_POINT('Ctrl Pts',(-16.6590249476465,-19.3718146562835,
-12.3343649558944));
#72112=CARTESIAN_POINT('Ctrl Pts',(-16.6607807173933,-19.3804012297473,
-12.3349028949872));
#72113=CARTESIAN_POINT('Ctrl Pts',(-16.6738381177958,-19.4422975436483,
-12.3388054876417));
#72114=CARTESIAN_POINT('Ctrl Pts',(-16.6871401814529,-19.4951596902494,
-12.3422714146459));
#72115=CARTESIAN_POINT('Ctrl Pts',(-16.710915326641,-19.5762756100903,-12.3477384364724));
#72116=CARTESIAN_POINT('Ctrl Pts',(-16.7199782499035,-19.6049225969443,
-12.3496987075554));
#72117=CARTESIAN_POINT('Ctrl Pts',(-16.7713467167216,-19.7560315446476,
-12.3601667422174));
#72118=CARTESIAN_POINT('Ctrl Pts',(-16.8242222547657,-19.8746197759884,
-12.3688106848789));
#72119=CARTESIAN_POINT('Ctrl Pts',(-16.9306835106997,-20.064426003423,-12.3828999435972));
#72120=CARTESIAN_POINT('Ctrl Pts',(-16.9785109570755,-20.1384668492301,
-12.3884748073271));
#72121=CARTESIAN_POINT('Ctrl Pts',(-17.0429913087979,-20.2258126884641,
-12.395137564478));
#72122=CARTESIAN_POINT('Ctrl Pts',(-17.0554044716555,-20.2421264502442,
-12.3963862245251));
#72123=CARTESIAN_POINT('Ctrl Pts',(-17.0735177871782,-20.2652274214933,
-12.3981610621399));
#72124=CARTESIAN_POINT('Ctrl Pts',(-17.0790263540612,-20.2721627455101,
-12.3986947835348));
#72125=CARTESIAN_POINT('Ctrl Pts',(-17.0886523388242,-20.2841269877132,
-12.399617127077));
#72126=CARTESIAN_POINT('Ctrl Pts',(-17.0927496603199,-20.289171851892,-12.4000065473993));
#72127=CARTESIAN_POINT('Ctrl Pts',(-17.1006731547311,-20.2988364399503,
-12.4007535785642));
#72128=CARTESIAN_POINT('Ctrl Pts',(-17.1044958522927,-20.303458920278,-12.401111324537));
#72129=CARTESIAN_POINT('Ctrl Pts',(-17.1145631269963,-20.3155276504802,
-12.4020465765252));
#72130=CARTESIAN_POINT('Ctrl Pts',(-17.1208394665978,-20.322947313913,-12.4026227815959));
#72131=CARTESIAN_POINT('Ctrl Pts',(-17.1428074041226,-20.3485572741231,
-12.4046161848513));
#72132=CARTESIAN_POINT('Ctrl Pts',(-17.1587577246184,-20.3665239270639,
-12.4060226930004));
#72133=CARTESIAN_POINT('Ctrl Pts',(-17.2748110920692,-20.4928498207702,
-12.4159804993574));
#72134=CARTESIAN_POINT('Ctrl Pts',(-17.3856945483354,-20.5907585268992,
-12.4240270587059));
#72135=CARTESIAN_POINT('Ctrl Pts',(-17.5439647497482,-20.7034829403172,
-12.4345796710768));
#72136=CARTESIAN_POINT('Ctrl Pts',(-17.5829479229916,-20.7293450426015,
-12.437116717034));
#72137=CARTESIAN_POINT('Ctrl Pts',(-17.6835103683468,-20.791362828888,-12.4435797683822));
#72138=CARTESIAN_POINT('Ctrl Pts',(-17.7461173731449,-20.8257316904768,
-12.4475293662063));
#72139=CARTESIAN_POINT('Ctrl Pts',(-17.8405408809355,-20.8715173157519,
-12.453547773292));
#72140=CARTESIAN_POINT('Ctrl Pts',(-17.8710889920245,-20.8854425849454,
-12.4555040949869));
#72141=CARTESIAN_POINT('Ctrl Pts',(-17.9086757220346,-20.9015082160251,
-12.4579375170801));
#72142=CARTESIAN_POINT('Ctrl Pts',(-17.9154129368002,-20.9043467070598,
-12.4583747109307));
#72143=CARTESIAN_POINT('Ctrl Pts',(-17.9259745501669,-20.9087321970095,
-12.4590618686022));
#72144=CARTESIAN_POINT('Ctrl Pts',(-17.9297890722405,-20.9103030412569,
-12.4593104118072));
#72145=CARTESIAN_POINT('Ctrl Pts',(-17.9369129639894,-20.9132123802894,
-12.4597753047112));
#72146=CARTESIAN_POINT('Ctrl Pts',(-17.9402211361437,-20.9145536574145,
-12.4599914832567));
#72147=CARTESIAN_POINT('Ctrl Pts',(-17.9477613383806,-20.9175886002641,
-12.4604848699888));
#72148=CARTESIAN_POINT('Ctrl Pts',(-17.9519954391431,-20.9192769617962,
-12.4607623921135));
#72149=CARTESIAN_POINT('Ctrl Pts',(-17.9630180965906,-20.9236310749426,
-12.4614860178304));
#72150=CARTESIAN_POINT('Ctrl Pts',(-17.9698149686861,-20.9262754178315,
-12.4619333569158));
#72151=CARTESIAN_POINT('Ctrl Pts',(-18.013180324473,-20.9428893497819,-12.4647940349285));
#72152=CARTESIAN_POINT('Ctrl Pts',(-18.0501142289988,-20.9558765461593,
-12.4672600161436));
#72153=CARTESIAN_POINT('Ctrl Pts',(-18.0991349441146,-20.9716008646714,
-12.4705524317999));
#72154=CARTESIAN_POINT('Ctrl Pts',(-18.1109183866702,-20.9752673041789,
-12.4713453165844));
#72155=CARTESIAN_POINT('Ctrl Pts',(-18.1458489787212,-20.98580193884,-12.4736987858701));
#72156=CARTESIAN_POINT('Ctrl Pts',(-18.1690819341408,-20.9923772854732,
-12.4752680532311));
#72157=CARTESIAN_POINT('Ctrl Pts',(-18.3317800649155,-21.0354320037361,
-12.4862637836891));
#72158=CARTESIAN_POINT('Ctrl Pts',(-18.4745550414503,-21.0579827035799,
-12.4959109169794));
#72159=CARTESIAN_POINT('Ctrl Pts',(-18.6802311550212,-21.0692194916129,
-12.509219179147));
#72160=CARTESIAN_POINT('Ctrl Pts',(-18.7420711558458,-21.0698870251877,
-12.5131507704253));
#72161=CARTESIAN_POINT('Ctrl Pts',(-18.8410951838317,-21.066617660406,-12.5193243928189));
#72162=CARTESIAN_POINT('Ctrl Pts',(-18.8782965839875,-21.0644052643062,
-12.5216163397455));
#72163=CARTESIAN_POINT('Ctrl Pts',(-18.9265161375305,-21.060257698663,-12.5245534348725));
#72164=CARTESIAN_POINT('Ctrl Pts',(-18.9376025876477,-21.0592159312481,
-12.525226415348));
#72165=CARTESIAN_POINT('Ctrl Pts',(-18.955614489402,-21.0573799178003,-12.5263161660786));
#72166=CARTESIAN_POINT('Ctrl Pts',(-18.9625450384991,-21.056638863885,-12.5267346022133));
#72167=CARTESIAN_POINT('Ctrl Pts',(-18.9758627008476,-21.0551483039326,
-12.5275370260485));
#72168=CARTESIAN_POINT('Ctrl Pts',(-18.9822502964348,-21.054403897001,-12.5279211696673));
#72169=CARTESIAN_POINT('Ctrl Pts',(-18.9968632835753,-21.0526333810973,
-12.5287983629214));
#72170=CARTESIAN_POINT('Ctrl Pts',(-19.005086272362,-21.051588041391,-12.5292908006172));
#72171=CARTESIAN_POINT('Ctrl Pts',(-19.0269054778989,-21.0486839738374,
-12.5305944562841));
#72172=CARTESIAN_POINT('Ctrl Pts',(-19.0404902626894,-21.0467412816943,
-12.5314030225098));
#72173=CARTESIAN_POINT('Ctrl Pts',(-19.1432878596563,-21.0310192693119,
-12.5374998570467));
#72174=CARTESIAN_POINT('Ctrl Pts',(-19.2315619172785,-21.011677809125,-12.542605636556));
#72175=CARTESIAN_POINT('Ctrl Pts',(-19.4524106042043,-20.9482546123032,
-12.5553256081018));
#72176=CARTESIAN_POINT('Ctrl Pts',(-19.5823413261859,-20.8965980082631,
-12.5627450703409));
#72177=CARTESIAN_POINT('Ctrl Pts',(-19.755360329122,-20.8071466963016,-12.5735038081901));
#72178=CARTESIAN_POINT('Ctrl Pts',(-19.8034593137398,-20.7798408335541,
-12.5766019163904));
#72179=CARTESIAN_POINT('Ctrl Pts',(-19.8746319555107,-20.7356645080236,
-12.5814338042496));
#72180=CARTESIAN_POINT('Ctrl Pts',(-19.8985260649091,-20.720157006408,-12.5831004506625));
#72181=CARTESIAN_POINT('Ctrl Pts',(-19.9278456863197,-20.7002762054967,
-12.5852110717727));
#72182=CARTESIAN_POINT('Ctrl Pts',(-19.9335733760471,-20.6963511475277,
-12.5856265638801));
#72183=CARTESIAN_POINT('Ctrl Pts',(-19.9426064176098,-20.6900954760322,
-12.5862870463402));
#72184=CARTESIAN_POINT('Ctrl Pts',(-19.9459246361934,-20.6877834058569,
-12.5865307918188));
#72185=CARTESIAN_POINT('Ctrl Pts',(-19.9521703936436,-20.6834048437636,
-12.5869917470716));
#72186=CARTESIAN_POINT('Ctrl Pts',(-19.955099318139,-20.6813404220923,-12.5872088162025));
#72187=CARTESIAN_POINT('Ctrl Pts',(-19.9617838667649,-20.6766034395958,
-12.5877062847042));
#72188=CARTESIAN_POINT('Ctrl Pts',(-19.9655360083536,-20.6739260456115,
-12.5879870134862));
#72189=CARTESIAN_POINT('Ctrl Pts',(-19.975474541165,-20.6667851638483,-12.5887345014587));
#72190=CARTESIAN_POINT('Ctrl Pts',(-19.9816455357087,-20.6623005021688,
-12.5892026657452));
#72191=CARTESIAN_POINT('Ctrl Pts',(-20.024702482516,-20.6306525913797,-12.5924967979107));
#72192=CARTESIAN_POINT('Ctrl Pts',(-20.0607196961468,-20.6023337784195,
-12.5953948294594));
#72193=CARTESIAN_POINT('Ctrl Pts',(-20.1245701968741,-20.5486893202651,
-12.6007562756045));
#72194=CARTESIAN_POINT('Ctrl Pts',(-20.1527030036379,-20.5237454690348,
-12.6032036500081));
#72195=CARTESIAN_POINT('Ctrl Pts',(-20.2758195357236,-20.4085850850627,
-12.6142537724694));
#72196=CARTESIAN_POINT('Ctrl Pts',(-20.36297939067,-20.3104098869636,-12.6229969641755));
#72197=CARTESIAN_POINT('Ctrl Pts',(-20.4927973386742,-20.1335789387884,
-12.6372014210681));
#72198=CARTESIAN_POINT('Ctrl Pts',(-20.5405828621735,-20.059139852871,-12.642796817856));
#72199=CARTESIAN_POINT('Ctrl Pts',(-20.5935715959742,-19.9639803495881,
-12.6494813230252));
#72200=CARTESIAN_POINT('Ctrl Pts',(-20.6033012857515,-19.9458931020195,
-12.6507323760418));
#72201=CARTESIAN_POINT('Ctrl Pts',(-20.6168513921819,-19.9198006994783,
-12.6525099853627));
#72202=CARTESIAN_POINT('Ctrl Pts',(-20.6208868722838,-19.9119091070977,
-12.6530441178926));
#72203=CARTESIAN_POINT('Ctrl Pts',(-20.6277957976667,-19.8981864137335,
-12.6539669434635));
#72204=CARTESIAN_POINT('Ctrl Pts',(-20.6306921440056,-19.8923670374509,
-12.654356436983));
#72205=CARTESIAN_POINT('Ctrl Pts',(-20.6362088784293,-19.8811535629588,
-12.6551034501763));
#72206=CARTESIAN_POINT('Ctrl Pts',(-20.6388332360704,-19.8757614977014,
-12.6554611057355));
#72207=CARTESIAN_POINT('Ctrl Pts',(-20.6456466878072,-19.8616099253851,
-12.6563957702967));
#72208=CARTESIAN_POINT('Ctrl Pts',(-20.6497985236599,-19.8528325576252,
-12.6569714815719));
#72209=CARTESIAN_POINT('Ctrl Pts',(-20.6639911323003,-19.8222861155732,
-12.6589614563516));
#72210=CARTESIAN_POINT('Ctrl Pts',(-20.6737226580472,-19.8003747830157,
-12.6603650794084));
#72211=CARTESIAN_POINT('Ctrl Pts',(-20.6971018432278,-19.7452280013232,
-12.6638422537416));
#72212=CARTESIAN_POINT('Ctrl Pts',(-20.7102719135608,-19.7118198044429,
-12.6658991664758));
#72213=CARTESIAN_POINT('Ctrl Pts',(-20.7225804971235,-19.6781106020849,
-12.6679319461521));
#72214=CARTESIAN_POINT('',(-20.8538228987003,-18.9509225630713,-11.6890562790225));
#72215=CARTESIAN_POINT('Ctrl Pts',(-20.7242504220745,-19.678735851896,-12.4443820803097));
#72216=CARTESIAN_POINT('Ctrl Pts',(-20.5136266400376,-20.2394180472743,
-12.4082724695729));
#72217=CARTESIAN_POINT('Ctrl Pts',(-19.519709855093,-21.2712729544138,-12.3297709232754));
#72218=CARTESIAN_POINT('Ctrl Pts',(-17.2597753208662,-20.9751143311526,
-12.2088774414178));
#72219=CARTESIAN_POINT('Ctrl Pts',(-16.2349111543522,-18.8074837620172,
-12.0817016347362));
#72220=CARTESIAN_POINT('Ctrl Pts',(-17.5028058927726,-16.7724378715414,
-11.9545258280549));
#72221=CARTESIAN_POINT('Ctrl Pts',(-19.9002448080497,-16.7370049550442,
-11.8273500213734));
#72222=CARTESIAN_POINT('Ctrl Pts',(-20.8239162058793,-18.1263146561008,
-11.7388601716959));
#72223=CARTESIAN_POINT('Ctrl Pts',(-20.8542040030872,-18.8895339278279,
-11.692762257579));
#72224=CARTESIAN_POINT('Ctrl Pts',(-20.8538228987003,-18.9509225630713,
-11.6890562790225));
#72225=CARTESIAN_POINT('Ctrl Pts',(-20.8509997772495,-18.951028853519,-11.6906773230242));
#72226=CARTESIAN_POINT('Ctrl Pts',(-20.8510794080773,-19.1246158951622,
-11.6795115293442));
#72227=CARTESIAN_POINT('Ctrl Pts',(-20.8298099013721,-19.2975644957165,
-11.6678002294521));
#72228=CARTESIAN_POINT('Ctrl Pts',(-20.7727929299519,-19.5253756648775,
-11.6526342526004));
#72229=CARTESIAN_POINT('Ctrl Pts',(-20.7553607601819,-19.5840902169118,
-11.6487420158878));
#72230=CARTESIAN_POINT('Ctrl Pts',(-20.7312404359986,-19.6540563010343,
-11.6441315496009));
#72231=CARTESIAN_POINT('Ctrl Pts',(-20.7269648807203,-19.6661031986997,
-11.6433386668622));
#72232=CARTESIAN_POINT('Ctrl Pts',(-20.7225805826898,-19.6781103677465,
-11.642549326843));
#72233=CARTESIAN_POINT('Origin',(-18.734,-18.952,0.));
#72234=CARTESIAN_POINT('',(-20.7225805823871,-19.6781103685755,-10.8441190550425));
#72235=CARTESIAN_POINT('',(-20.7225805818558,-19.6781103700305,-11.0644159698366));
#72236=CARTESIAN_POINT('',(-20.7225805821191,-19.6781103693095,0.));
#72237=CARTESIAN_POINT('Ctrl Pts',(-20.7225805818558,-19.6781103700305,
-11.0644159698366));
#72238=CARTESIAN_POINT('Ctrl Pts',(-20.7579844873321,-19.5811505663178,
-11.0708124775531));
#72239=CARTESIAN_POINT('Ctrl Pts',(-20.7862468792086,-19.4817385396693,
-11.0775607479106));
#72240=CARTESIAN_POINT('Ctrl Pts',(-20.8362075101163,-19.2401187738218,
-11.0938352048317));
#72241=CARTESIAN_POINT('Ctrl Pts',(-20.850904768817,-19.0969559230897,-11.1033538061458));
#72242=CARTESIAN_POINT('Ctrl Pts',(-20.8510404642511,-18.8914033906172,
-11.1164064283306));
#72243=CARTESIAN_POINT('Ctrl Pts',(-20.8483582573918,-18.8294329440592,
-11.1202674706854));
#72244=CARTESIAN_POINT('Ctrl Pts',(-20.8418780036,-18.7552932863852,-11.1248002585708));
#72245=CARTESIAN_POINT('Ctrl Pts',(-20.8406878626443,-18.7429319035788,
-11.1255531701033));
#72246=CARTESIAN_POINT('Ctrl Pts',(-20.8385539133076,-18.7226409458399,
-11.1267845412211));
#72247=CARTESIAN_POINT('Ctrl Pts',(-20.8376739010565,-18.7147050980675,
-11.1272649965875));
#72248=CARTESIAN_POINT('Ctrl Pts',(-20.8360103029312,-18.7004401585787,
-11.1281266408321));
#72249=CARTESIAN_POINT('Ctrl Pts',(-20.8352429789031,-18.6941093013817,
-11.128508337234));
#72250=CARTESIAN_POINT('Ctrl Pts',(-20.8335469916613,-18.6806267574853,
-11.1293197527859));
#72251=CARTESIAN_POINT('Ctrl Pts',(-20.8326103660227,-18.673476140081,-11.1297492155852));
#72252=CARTESIAN_POINT('Ctrl Pts',(-20.829987445343,-18.6542163531508,-11.1309036536396));
#72253=CARTESIAN_POINT('Ctrl Pts',(-20.8282327463475,-18.6421166591405,
-11.1316264622143));
#72254=CARTESIAN_POINT('Ctrl Pts',(-20.8189028629222,-18.581484427413,-11.1352369958233));
#72255=CARTESIAN_POINT('Ctrl Pts',(-20.8097446721144,-18.5332084702202,
-11.1380742019443));
#72256=CARTESIAN_POINT('Ctrl Pts',(-20.77842894594,-18.3946544175901,-11.1461498406355));
#72257=CARTESIAN_POINT('Ctrl Pts',(-20.7519967217578,-18.3054591454402,
-11.1512604423142));
#72258=CARTESIAN_POINT('Ctrl Pts',(-20.662349994649,-18.0628319145366,-11.1653489677555));
#72259=CARTESIAN_POINT('Ctrl Pts',(-20.5868669751842,-17.9146859160175,
-11.1741494194995));
#72260=CARTESIAN_POINT('Ctrl Pts',(-20.4871421882956,-17.7652493966157,
-11.18471080089));
#72261=CARTESIAN_POINT('Ctrl Pts',(-20.4792655345325,-17.7536958993347,
-11.18553946098));
#72262=CARTESIAN_POINT('Ctrl Pts',(-20.4681194465743,-17.737689808394,-11.1867057626787));
#72263=CARTESIAN_POINT('Ctrl Pts',(-20.4649459669798,-17.733170416235,-11.1870371320656));
#72264=CARTESIAN_POINT('Ctrl Pts',(-20.4598136868389,-17.7259219425457,
-11.1875720124777));
#72265=CARTESIAN_POINT('Ctrl Pts',(-20.4578659848135,-17.7231849810935,
-11.1877747655506));
#72266=CARTESIAN_POINT('Ctrl Pts',(-20.453774816735,-17.7174648349837,-11.1882001881634));
#72267=CARTESIAN_POINT('Ctrl Pts',(-20.4516300983818,-17.7144825906876,
-11.1884229470425));
#72268=CARTESIAN_POINT('Ctrl Pts',(-20.4464076162279,-17.7072604265331,
-11.1889647147434));
#72269=CARTESIAN_POINT('Ctrl Pts',(-20.4433218642617,-17.7030263361959,
-11.1892842714886));
#72270=CARTESIAN_POINT('Ctrl Pts',(-20.4323912721032,-17.6881443887543,
-11.1904141674171));
#72271=CARTESIAN_POINT('Ctrl Pts',(-20.4244625858972,-17.6775588893136,
-11.1912300439275));
#72272=CARTESIAN_POINT('Ctrl Pts',(-20.3764348900314,-17.6146744062217,
-11.1961467917197));
#72273=CARTESIAN_POINT('Ctrl Pts',(-20.3340141529888,-17.564201330716,-11.2003845261687));
#72274=CARTESIAN_POINT('Ctrl Pts',(-20.2240817521247,-17.4451520266549,
-11.2109621644093));
#72275=CARTESIAN_POINT('Ctrl Pts',(-20.1541137412452,-17.3790374347441,
-11.2173578349685));
#72276=CARTESIAN_POINT('Ctrl Pts',(-19.9712621129894,-17.2284345051613,
-11.2329413739918));
#72277=CARTESIAN_POINT('Ctrl Pts',(-19.8539618884946,-17.1500027207405,
-11.2419899121193));
#72278=CARTESIAN_POINT('Ctrl Pts',(-19.7171140998958,-17.0770653795885,
-11.2514585608735));
#72279=CARTESIAN_POINT('Ctrl Pts',(-19.7044367136208,-17.0704724916167,
-11.2523264913288));
#72280=CARTESIAN_POINT('Ctrl Pts',(-19.6841535537,-17.0601837564007,-11.2537007415871));
#72281=CARTESIAN_POINT('Ctrl Pts',(-19.676590880354,-17.0564043388244,-11.2542099890717));
#72282=CARTESIAN_POINT('Ctrl Pts',(-19.6632128771048,-17.0498185896777,
-11.2551053519251));
#72283=CARTESIAN_POINT('Ctrl Pts',(-19.6574070065859,-17.0469933883648,
-11.2554921233506));
#72284=CARTESIAN_POINT('Ctrl Pts',(-19.6453717582343,-17.041204850674,-11.2562901949485));
#72285=CARTESIAN_POINT('Ctrl Pts',(-19.6391406328896,-17.038245308087,-11.2567013597033));
#72286=CARTESIAN_POINT('Ctrl Pts',(-19.6231088304744,-17.0307266402043,
-11.2577540977608));
#72287=CARTESIAN_POINT('Ctrl Pts',(-19.6132874240169,-17.0262119877792,
-11.2583941295991));
#72288=CARTESIAN_POINT('Ctrl Pts',(-19.5721500402048,-17.0076824878413,
-11.2610550190411));
#72289=CARTESIAN_POINT('Ctrl Pts',(-19.5405292519066,-16.9943542607359,
-11.2630523428465));
#72290=CARTESIAN_POINT('Ctrl Pts',(-19.4573061818126,-16.96163456475,-11.2681970385183));
#72291=CARTESIAN_POINT('Ctrl Pts',(-19.4052450622355,-16.9434788747606,
-11.2713050089752));
#72292=CARTESIAN_POINT('Ctrl Pts',(-19.2479505595839,-16.8954247313737,
-11.2804501372988));
#72293=CARTESIAN_POINT('Ctrl Pts',(-19.1410481911417,-16.8716251140253,
-11.2863385681661));
#72294=CARTESIAN_POINT('Ctrl Pts',(-18.9869106877308,-16.8496507161838,
-11.294815342171));
#72295=CARTESIAN_POINT('Ctrl Pts',(-18.9408341897008,-16.8446187586796,
-11.2973492262774));
#72296=CARTESIAN_POINT('Ctrl Pts',(-18.8732968578577,-16.8394794261704,
-11.3011064623954));
#72297=CARTESIAN_POINT('Ctrl Pts',(-18.8519396268359,-16.8381795272402,
-11.3023009260558));
#72298=CARTESIAN_POINT('Ctrl Pts',(-18.7787678745559,-16.8348383223842,
-11.3064254654049));
#72299=CARTESIAN_POINT('Ctrl Pts',(-18.7269038955648,-16.8343771739595,
-11.3094040309555));
#72300=CARTESIAN_POINT('Ctrl Pts',(-18.6664282352558,-16.8360609722037,
-11.3129946951207));
#72301=CARTESIAN_POINT('Ctrl Pts',(-18.6577780991352,-16.8363549142684,
-11.3135110982405));
#72302=CARTESIAN_POINT('Ctrl Pts',(-18.6446645621392,-16.8368810545605,
-11.3142985533844));
#72303=CARTESIAN_POINT('Ctrl Pts',(-18.6401995732535,-16.8370743623204,
-11.3145674793427));
#72304=CARTESIAN_POINT('Ctrl Pts',(-18.6321760289926,-16.8374471927784,
-11.3150522420014));
#72305=CARTESIAN_POINT('Ctrl Pts',(-18.628617288541,-16.8376215619198,-11.3152677873554));
#72306=CARTESIAN_POINT('Ctrl Pts',(-18.6208737562566,-16.8380205735515,
-11.315737972356));
#72307=CARTESIAN_POINT('Ctrl Pts',(-18.6166892399142,-16.8382486552726,
-11.3159927972084));
#72308=CARTESIAN_POINT('Ctrl Pts',(-18.6049071606807,-16.838925944523,-11.3167123292818));
#72309=CARTESIAN_POINT('Ctrl Pts',(-18.597311393328,-16.8394036954825,-11.3171785901851));
#72310=CARTESIAN_POINT('Ctrl Pts',(-18.551291574423,-16.8425474286557,-11.3200172816168));
#72311=CARTESIAN_POINT('Ctrl Pts',(-18.512946147429,-16.8462205047304,-11.32244082374));
#72312=CARTESIAN_POINT('Ctrl Pts',(-18.3856261185697,-16.8619320178184,
-11.3306360958104));
#72313=CARTESIAN_POINT('Ctrl Pts',(-18.297322067007,-16.8785827890315,-11.3365589563103));
#72314=CARTESIAN_POINT('Ctrl Pts',(-18.0441406902274,-16.9432172183882,
-11.3538259097801));
#72315=CARTESIAN_POINT('Ctrl Pts',(-17.883673604404,-17.0057006591603,-11.3650719540722));
#72316=CARTESIAN_POINT('Ctrl Pts',(-17.7119985427835,-17.097884859132,-11.3770690553889));
#72317=CARTESIAN_POINT('Ctrl Pts',(-17.6916899067312,-17.1092250079467,
-11.3784891185983));
#72318=CARTESIAN_POINT('Ctrl Pts',(-17.6632766092955,-17.1257107591034,
-11.3804778074892));
#72319=CARTESIAN_POINT('Ctrl Pts',(-17.6550142981273,-17.130579996073,-11.381056335434));
#72320=CARTESIAN_POINT('Ctrl Pts',(-17.6416585665028,-17.1385737150611,
-11.3819919745945));
#72321=CARTESIAN_POINT('Ctrl Pts',(-17.6365448535094,-17.141663870763,-11.3823503299366));
#72322=CARTESIAN_POINT('Ctrl Pts',(-17.6258802996449,-17.1481701272996,
-11.3830979400449));
#72323=CARTESIAN_POINT('Ctrl Pts',(-17.6203320074089,-17.1515903011523,
-11.3834870404065));
#72324=CARTESIAN_POINT('Ctrl Pts',(-17.6071925293078,-17.1597739433391,
-11.3844089199815));
#72325=CARTESIAN_POINT('Ctrl Pts',(-17.5996155826525,-17.1645601236342,
-11.3849408545199));
#72326=CARTESIAN_POINT('Ctrl Pts',(-17.5742946242304,-17.1807806392733,
-11.3867198010634));
#72327=CARTESIAN_POINT('Ctrl Pts',(-17.5566909265376,-17.1924324464752,
-11.3879587166515));
#72328=CARTESIAN_POINT('Ctrl Pts',(-17.4624627602254,-17.2568489618403,
-11.3946071354624));
#72329=CARTESIAN_POINT('Ctrl Pts',(-17.3892011751445,-17.3143605354946,
-11.3998310507177));
#72330=CARTESIAN_POINT('Ctrl Pts',(-17.2048037462984,-17.4798624873552,
-11.4134760685261));
#72331=CARTESIAN_POINT('Ctrl Pts',(-17.1013405781946,-17.595516747048,-11.4216583478927));
#72332=CARTESIAN_POINT('Ctrl Pts',(-16.9802309195438,-17.7650459394442,
-11.433372371975));
#72333=CARTESIAN_POINT('Ctrl Pts',(-16.9507247510517,-17.8098554024099,
-11.436449435185));
#72334=CARTESIAN_POINT('Ctrl Pts',(-16.9184277827835,-17.8632103356466,
-11.4401504167748));
#72335=CARTESIAN_POINT('Ctrl Pts',(-16.9139476690044,-17.8707160800193,
-11.4406718866123));
#72336=CARTESIAN_POINT('Ctrl Pts',(-16.9072380496975,-17.8821168676759,
-11.4414655587312));
#72337=CARTESIAN_POINT('Ctrl Pts',(-16.9049741730571,-17.8859917151222,
-11.4417355842843));
#72338=CARTESIAN_POINT('Ctrl Pts',(-16.9009344145529,-17.8929569113979,
-11.4422215142728));
#72339=CARTESIAN_POINT('Ctrl Pts',(-16.8991540024281,-17.8960445705582,
-11.4424371210916));
#72340=CARTESIAN_POINT('Ctrl Pts',(-16.895304288382,-17.9027600262537,-11.4429064864137));
#72341=CARTESIAN_POINT('Ctrl Pts',(-16.8932379489929,-17.906389406468,-11.4431604249098));
#72342=CARTESIAN_POINT('Ctrl Pts',(-16.8874688996558,-17.9165924383327,
-11.4438750071541));
#72343=CARTESIAN_POINT('Ctrl Pts',(-16.8837906155752,-17.9231797274809,
-11.4443371712664));
#72344=CARTESIAN_POINT('Ctrl Pts',(-16.8621105825172,-17.962497909465,-11.4470999244142));
#72345=CARTESIAN_POINT('Ctrl Pts',(-16.8449436796381,-17.9956788191202,
-11.4494485653246));
#72346=CARTESIAN_POINT('Ctrl Pts',(-16.7915437151275,-18.1059466968339,
-11.4572675946221));
#72347=CARTESIAN_POINT('Ctrl Pts',(-16.7590845511968,-18.1847648905646,
-11.4628754206623));
#72348=CARTESIAN_POINT('Ctrl Pts',(-16.6736958740607,-18.4337796735083,
-11.4802659812416));
#72349=CARTESIAN_POINT('Ctrl Pts',(-16.6374055860073,-18.6088939673275,
-11.4919694303881));
#72350=CARTESIAN_POINT('Ctrl Pts',(-16.6216971068866,-18.8092250006362,
-11.5043355398657));
#72351=CARTESIAN_POINT('Ctrl Pts',(-16.6202826718643,-18.8319694491984,
-11.5057263784402));
#72352=CARTESIAN_POINT('Ctrl Pts',(-16.6187986224762,-18.8642354321953,
-11.5076815417981));
#72353=CARTESIAN_POINT('Ctrl Pts',(-16.6184256124905,-18.8737408000677,
-11.5082553233971));
#72354=CARTESIAN_POINT('Ctrl Pts',(-16.6179230993141,-18.8892060477199,
-11.5091853748408));
#72355=CARTESIAN_POINT('Ctrl Pts',(-16.6177546806795,-18.8951644508896,
-11.5095428596705));
#72356=CARTESIAN_POINT('Ctrl Pts',(-16.6174544999128,-18.9076515434461,
-11.5102903092406));
#72357=CARTESIAN_POINT('Ctrl Pts',(-16.6173277742421,-18.9141802998865,
-11.5106801123024));
#72358=CARTESIAN_POINT('Ctrl Pts',(-16.6170977999836,-18.92973785894,-11.5116066667348));
#72359=CARTESIAN_POINT('Ctrl Pts',(-16.6170221024747,-18.9387669884501,
-11.5121425500491));
#72360=CARTESIAN_POINT('Ctrl Pts',(-16.616961468523,-18.9693033990417,-11.513948816493));
#72361=CARTESIAN_POINT('Ctrl Pts',(-16.6172465045199,-18.9908103195865,
-11.5152107542175));
#72362=CARTESIAN_POINT('Ctrl Pts',(-16.6229840477437,-19.1921284540706,
-11.5269368435748));
#72363=CARTESIAN_POINT('Ctrl Pts',(-16.6510054389155,-19.3705577992118,
-11.5365998245621));
#72364=CARTESIAN_POINT('Ctrl Pts',(-16.7347789666902,-19.6585463785539,
-11.5529241017152));
#72365=CARTESIAN_POINT('Ctrl Pts',(-16.7780349048173,-19.7707091566606,
-11.5595103938139));
#72366=CARTESIAN_POINT('Ctrl Pts',(-16.8347118640321,-19.8871385202989,
-11.5671846549436));
#72367=CARTESIAN_POINT('Ctrl Pts',(-16.8389326008756,-19.8956625565929,
-11.5677516144617));
#72368=CARTESIAN_POINT('Ctrl Pts',(-16.8452721866534,-19.9082516709598,
-11.5685969769487));
#72369=CARTESIAN_POINT('Ctrl Pts',(-16.84734709472,-19.9123389116424,-11.5688726978324));
#72370=CARTESIAN_POINT('Ctrl Pts',(-16.8510625607891,-19.9195992766697,
-11.5693647795511));
#72371=CARTESIAN_POINT('Ctrl Pts',(-16.8526978919293,-19.922775019319,-11.5695808104175));
#72372=CARTESIAN_POINT('Ctrl Pts',(-16.8562312901945,-19.9295942664112,
-11.5700464092219));
#72373=CARTESIAN_POINT('Ctrl Pts',(-16.8581318996417,-19.9332363357724,
-11.5702961320384));
#72374=CARTESIAN_POINT('Ctrl Pts',(-16.8634079138655,-19.9432752191973,
-11.5709873215845));
#72375=CARTESIAN_POINT('Ctrl Pts',(-16.8668054815038,-19.9496602325058,
-11.5714301556311));
#72376=CARTESIAN_POINT('Ctrl Pts',(-16.8856059253174,-19.9845592700827,
-11.5738677463297));
#72377=CARTESIAN_POINT('Ctrl Pts',(-16.9016284040048,-20.012732468425,-11.5758985539128));
#72378=CARTESIAN_POINT('Ctrl Pts',(-17.0020051347757,-20.1801654887417,
-11.5883018036747));
#72379=CARTESIAN_POINT('Ctrl Pts',(-17.1015465148793,-20.3096789800685,
-11.5992662296815));
#72380=CARTESIAN_POINT('Ctrl Pts',(-17.2963442641619,-20.5103622226945,
-11.6175348600792));
#72381=CARTESIAN_POINT('Ctrl Pts',(-17.3845566913055,-20.5873462648025,
-11.6249792661696));
#72382=CARTESIAN_POINT('Ctrl Pts',(-17.4901846040866,-20.6651305013763,
-11.6329888615444));
#72383=CARTESIAN_POINT('Ctrl Pts',(-17.5017669852199,-20.6734803707338,
-11.6338561231333));
#72384=CARTESIAN_POINT('Ctrl Pts',(-17.5203382624236,-20.686585140214,-11.6352295178388));
#72385=CARTESIAN_POINT('Ctrl Pts',(-17.5272725358787,-20.691416353976,-11.6357385729682));
#72386=CARTESIAN_POINT('Ctrl Pts',(-17.539554898624,-20.6998648637377,-11.6366337121068));
#72387=CARTESIAN_POINT('Ctrl Pts',(-17.5448909187911,-20.7034994366282,
-11.6370204511408));
#72388=CARTESIAN_POINT('Ctrl Pts',(-17.5559635325566,-20.7109675049447,
-11.6378185655833));
#72389=CARTESIAN_POINT('Ctrl Pts',(-17.5617024134304,-20.7147974847763,
-11.6382298050335));
#72390=CARTESIAN_POINT('Ctrl Pts',(-17.5764847992254,-20.7245587498564,
-11.6392829614986));
#72391=CARTESIAN_POINT('Ctrl Pts',(-17.5855552873038,-20.7304489619235,
-11.639923334643));
#72392=CARTESIAN_POINT('Ctrl Pts',(-17.6236297688466,-20.7547610822365,
-11.6425875437171));
#72393=CARTESIAN_POINT('Ctrl Pts',(-17.6530358950941,-20.772545624605,-11.6445877708354));
#72394=CARTESIAN_POINT('Ctrl Pts',(-17.7307999031055,-20.8170277141788,
-11.6497416379285));
#72395=CARTESIAN_POINT('Ctrl Pts',(-17.7797933692674,-20.8425631869656,
-11.65285569201));
#72396=CARTESIAN_POINT('Ctrl Pts',(-18.0003559669081,-20.9467593781062,
-11.6664180841387));
#72397=CARTESIAN_POINT('Ctrl Pts',(-18.1809676349705,-21.0041792710223,
-11.6762656388817));
#72398=CARTESIAN_POINT('Ctrl Pts',(-18.4073602201613,-21.0440548965402,
-11.6893368017394));
#72399=CARTESIAN_POINT('Ctrl Pts',(-18.4481422604152,-21.0500162262898,
-11.6917225301682));
#72400=CARTESIAN_POINT('Ctrl Pts',(-18.4964149175663,-21.055638995056,-11.6946101484542));
#72401=CARTESIAN_POINT('Ctrl Pts',(-18.5037650309882,-21.0564561169903,
-11.6950515590223));
#72402=CARTESIAN_POINT('Ctrl Pts',(-18.5156829041899,-21.0577178602441,
-11.695770313428));
#72403=CARTESIAN_POINT('Ctrl Pts',(-18.5202481653399,-21.0581861773223,
-11.6960463585453));
#72404=CARTESIAN_POINT('Ctrl Pts',(-18.5283700476443,-21.0589926641191,
-11.6965387953529));
#72405=CARTESIAN_POINT('Ctrl Pts',(-18.5319260380648,-21.0593366787582,
-11.6967548552368));
#72406=CARTESIAN_POINT('Ctrl Pts',(-18.5395694361031,-21.0600565939946,
-11.6972202617655));
#72407=CARTESIAN_POINT('Ctrl Pts',(-18.5436570107701,-21.0604296036271,
-11.6974697619459));
#72408=CARTESIAN_POINT('Ctrl Pts',(-18.5549340111549,-21.0614256203844,
-11.6981597224047));
#72409=CARTESIAN_POINT('Ctrl Pts',(-18.5621254989973,-21.0620237507538,
-11.6986015421587));
#72410=CARTESIAN_POINT('Ctrl Pts',(-18.6013929219655,-21.0650876251846,
-11.7010234222429));
#72411=CARTESIAN_POINT('Ctrl Pts',(-18.6335169706994,-21.0668585884061,
-11.703038998777));
#72412=CARTESIAN_POINT('Ctrl Pts',(-18.8285955317185,-21.0731586812053,
-11.7154371960103));
#72413=CARTESIAN_POINT('Ctrl Pts',(-18.9915820964966,-21.0595848288149,
-11.7264156691741));
#72414=CARTESIAN_POINT('Ctrl Pts',(-19.2659917298223,-21.0043979204939,
-11.7446994764501));
#72415=CARTESIAN_POINT('Ctrl Pts',(-19.3784964379381,-20.9718971723678,
-11.7521456795152));
#72416=CARTESIAN_POINT('Ctrl Pts',(-19.5011222370866,-20.9251743462991,
-11.7601584202365));
#72417=CARTESIAN_POINT('Ctrl Pts',(-19.5144346470234,-20.9199469771841,
-11.7610271329673));
#72418=CARTESIAN_POINT('Ctrl Pts',(-19.5355343766359,-20.9114139890556,
-11.7624023837635));
#72419=CARTESIAN_POINT('Ctrl Pts',(-19.5433564412223,-20.9081959747764,
-11.762911856147));
#72420=CARTESIAN_POINT('Ctrl Pts',(-19.5571159429487,-20.902438627853,-11.7638074806225));
#72421=CARTESIAN_POINT('Ctrl Pts',(-19.5630614014326,-20.8999188614121,
-11.7641942899779));
#72422=CARTESIAN_POINT('Ctrl Pts',(-19.5744705594249,-20.8950218064413,
-11.7649362382588));
#72423=CARTESIAN_POINT('Ctrl Pts',(-19.5799359258969,-20.8926485802329,
-11.7652915109602));
#72424=CARTESIAN_POINT('Ctrl Pts',(-19.5943402722727,-20.8863213676107,
-11.7662275147921));
#72425=CARTESIAN_POINT('Ctrl Pts',(-19.6032620811115,-20.8823284633698,
-11.7668069104198));
#72426=CARTESIAN_POINT('Ctrl Pts',(-19.6363021087377,-20.8672660674517,
-11.768951572079));
#72427=CARTESIAN_POINT('Ctrl Pts',(-19.6602398224105,-20.8558048977944,
-11.7705033494632));
#72428=CARTESIAN_POINT('Ctrl Pts',(-19.7190620055048,-20.8262691787175,
-11.7743162838781));
#72429=CARTESIAN_POINT('Ctrl Pts',(-19.7536713989744,-20.8076676992583,
-11.7765593758584));
#72430=CARTESIAN_POINT('Ctrl Pts',(-19.8816292581679,-20.7342327264881,
-11.7848832307175));
#72431=CARTESIAN_POINT('Ctrl Pts',(-19.9712475386277,-20.6732283674483,
-11.7907667202882));
#72432=CARTESIAN_POINT('Ctrl Pts',(-20.1621981724831,-20.5205947240546,
-11.8040419224601));
#72433=CARTESIAN_POINT('Ctrl Pts',(-20.2601175449013,-20.4254973343465,
-11.8113990711624));
#72434=CARTESIAN_POINT('Ctrl Pts',(-20.3583114625171,-20.3097720358783,
-11.8202987225759));
#72435=CARTESIAN_POINT('Ctrl Pts',(-20.3682777801224,-20.2977595379688,
-11.8212221183077));
#72436=CARTESIAN_POINT('Ctrl Pts',(-20.3817499136355,-20.2811510848299,
-11.8224999853794));
#72437=CARTESIAN_POINT('Ctrl Pts',(-20.3853713640904,-20.2766490102178,
-11.8228464956567));
#72438=CARTESIAN_POINT('Ctrl Pts',(-20.391099894762,-20.269467478861,-11.8233995229171));
#72439=CARTESIAN_POINT('Ctrl Pts',(-20.3932190424407,-20.2667976224114,
-11.8236051829998));
#72440=CARTESIAN_POINT('Ctrl Pts',(-20.3975850636709,-20.2612696259498,
-11.824031163451));
#72441=CARTESIAN_POINT('Ctrl Pts',(-20.3998310193153,-20.2584108204592,
-11.8242515487345));
#72442=CARTESIAN_POINT('Ctrl Pts',(-20.4051694706375,-20.2515795261911,
-11.8247783612546));
#72443=CARTESIAN_POINT('Ctrl Pts',(-20.408255171997,-20.2476017761356,-11.8250852652578));
#72444=CARTESIAN_POINT('Ctrl Pts',(-20.418634009445,-20.2341235137528,-11.8261255781667));
#72445=CARTESIAN_POINT('Ctrl Pts',(-20.4258605442536,-20.2245723295287,
-11.8268634411502));
#72446=CARTESIAN_POINT('Ctrl Pts',(-20.5082067674954,-20.1137955701971,
-11.8354239296354));
#72447=CARTESIAN_POINT('Ctrl Pts',(-20.5742144263623,-20.0061265644406,
-11.8437541602859));
#72448=CARTESIAN_POINT('Ctrl Pts',(-20.6639559109624,-19.8253310612981,
-11.8570928881668));
#72449=CARTESIAN_POINT('Ctrl Pts',(-20.6939932569247,-19.7556568638507,
-11.862096629707));
#72450=CARTESIAN_POINT('Ctrl Pts',(-20.7210162224442,-19.6823839466691,
-11.8671696830208));
#72451=CARTESIAN_POINT('Ctrl Pts',(-20.7218001284805,-19.6802477784641,
-11.8673174213476));
#72452=CARTESIAN_POINT('Ctrl Pts',(-20.7225805820713,-19.6781103694405,
-11.8674650853572));
#72453=CARTESIAN_POINT('Ctrl Pts',(-20.7225805826898,-19.6781103677465,
-11.642549326843));
#72454=CARTESIAN_POINT('Ctrl Pts',(-20.7142737541329,-19.7008600745484,
-11.6410537824784));
#72455=CARTESIAN_POINT('Ctrl Pts',(-20.7055765608164,-19.7234671650752,
-11.6395709790409));
#72456=CARTESIAN_POINT('Ctrl Pts',(-20.6923270196944,-19.7562186672103,
-11.6374269988322));
#72457=CARTESIAN_POINT('Ctrl Pts',(-20.6880803544136,-19.7664828768096,
-11.6367556865579));
#72458=CARTESIAN_POINT('Ctrl Pts',(-20.6810401204349,-19.7831271056101,
-11.6356679616845));
#72459=CARTESIAN_POINT('Ctrl Pts',(-20.6782955490836,-19.7895275015664,
-11.6352498947636));
#72460=CARTESIAN_POINT('Ctrl Pts',(-20.6729551092705,-19.8018137818539,
-11.6344477271332));
#72461=CARTESIAN_POINT('Ctrl Pts',(-20.670363901434,-19.8077015964858,-11.6340634729269));
#72462=CARTESIAN_POINT('Ctrl Pts',(-20.6643671010903,-19.8211609627361,
-11.6331854006886));
#72463=CARTESIAN_POINT('Ctrl Pts',(-20.6609437117122,-19.8287245057633,
-11.6326921988427));
#72464=CARTESIAN_POINT('Ctrl Pts',(-20.6517254935704,-19.8487761465608,
-11.6313851760237));
#72465=CARTESIAN_POINT('Ctrl Pts',(-20.645853133331,-19.8612283187725,-11.6305740289688));
#72466=CARTESIAN_POINT('Ctrl Pts',(-20.5998122863577,-19.9564380024344,
-11.6243741118654));
#72467=CARTESIAN_POINT('Ctrl Pts',(-20.554407193293,-20.0365606683844,-11.6191752932871));
#72468=CARTESIAN_POINT('Ctrl Pts',(-20.4267062017835,-20.2311580598958,
-11.6063012206764));
#72469=CARTESIAN_POINT('Ctrl Pts',(-20.3379453853446,-20.3408328134021,
-11.5988194733751));
#72470=CARTESIAN_POINT('Ctrl Pts',(-20.201614149999,-20.4786360478685,-11.5880939164555));
#72471=CARTESIAN_POINT('Ctrl Pts',(-20.162862190324,-20.5149654463813,-11.5851129140871));
#72472=CARTESIAN_POINT('Ctrl Pts',(-20.1088879984315,-20.5618792481894,
-11.5809842414364));
#72473=CARTESIAN_POINT('Ctrl Pts',(-20.0948309131645,-20.5737790789704,
-11.5799109528858));
#72474=CARTESIAN_POINT('Ctrl Pts',(-20.0738433234799,-20.5910808464022,
-11.578308355089));
#72475=CARTESIAN_POINT('Ctrl Pts',(-20.0670312092362,-20.5966257756623,
-11.5777881635711));
#72476=CARTESIAN_POINT('Ctrl Pts',(-20.0546983476196,-20.6065375246519,
-11.5768459455248));
#72477=CARTESIAN_POINT('Ctrl Pts',(-20.0491899118001,-20.6109195395256,
-11.5764249479618));
#72478=CARTESIAN_POINT('Ctrl Pts',(-20.0404619766761,-20.6177919047249,
-11.5757574586586));
#72479=CARTESIAN_POINT('Ctrl Pts',(-20.0372569157665,-20.6203006255508,
-11.5755122528289));
#72480=CARTESIAN_POINT('Ctrl Pts',(-20.0340353601645,-20.622807308597,-11.5752656712314));
#72481=CARTESIAN_POINT('Ctrl Pts',(-20.0340260484216,-20.6228145539121,
-11.5752649584989));
#72482=CARTESIAN_POINT('Ctrl Pts',(-20.0340073890624,-20.6228290722044,
-11.5752635302861));
#72483=CARTESIAN_POINT('Ctrl Pts',(-20.0339980418306,-20.6228363448815,
-11.5752628148353));
#72484=CARTESIAN_POINT('Ctrl Pts',(-20.0339793113038,-20.6228509180425,
-11.5752613811714));
#72485=CARTESIAN_POINT('Ctrl Pts',(-20.0339699277046,-20.6228582187622,
-11.575260662935));
#72486=CARTESIAN_POINT('Ctrl Pts',(-20.0339511244705,-20.6228728479841,
-11.5752592237021));
#72487=CARTESIAN_POINT('Ctrl Pts',(-20.0339417043797,-20.62288017684,-11.5752585026707));
#72488=CARTESIAN_POINT('Ctrl Pts',(-20.0339228272802,-20.6228948630179,
-11.5752570577801));
#72489=CARTESIAN_POINT('Ctrl Pts',(-20.0339133707563,-20.6229022199615,
-11.575256333958));
#72490=CARTESIAN_POINT('Ctrl Pts',(-20.0338936955076,-20.6229175265545,
-11.5752548279714));
#72491=CARTESIAN_POINT('Ctrl Pts',(-20.0338834764892,-20.6229254764106,
-11.5752540457842));
#72492=CARTESIAN_POINT('Ctrl Pts',(-20.0338628599782,-20.6229415146626,
-11.5752524677467));
#72493=CARTESIAN_POINT('Ctrl Pts',(-20.0338524628754,-20.62294960275,-11.5752516719262));
#72494=CARTESIAN_POINT('Ctrl Pts',(-20.0338314864396,-20.6229659203706,
-11.5752500663343));
#72495=CARTESIAN_POINT('Ctrl Pts',(-20.0338209071046,-20.6229741498998,
-11.5752492565628));
#72496=CARTESIAN_POINT('Ctrl Pts',(-20.0337995625962,-20.6229907531943,
-11.5752476227927));
#72497=CARTESIAN_POINT('Ctrl Pts',(-20.0337887971895,-20.6229991271353,
-11.5752467987762));
#72498=CARTESIAN_POINT('Ctrl Pts',(-20.0337670763489,-20.6230160224941,
-11.5752451361955));
#72499=CARTESIAN_POINT('Ctrl Pts',(-20.0337561210846,-20.6230245437742,
-11.5752442976441));
#72500=CARTESIAN_POINT('Ctrl Pts',(-20.0337340164851,-20.6230417369387,
-11.5752426056839));
#72501=CARTESIAN_POINT('Ctrl Pts',(-20.0337228670254,-20.6230504089137,
-11.5752417522654));
#72502=CARTESIAN_POINT('Ctrl Pts',(-20.0337003696859,-20.6230679068323,
-11.575240030238));
#72503=CARTESIAN_POINT('Ctrl Pts',(-20.0336890220284,-20.6230767325965,
-11.575239161646));
#72504=CARTESIAN_POINT('Ctrl Pts',(-20.0336661241077,-20.6230945413294,
-11.575237408951));
#72505=CARTESIAN_POINT('Ctrl Pts',(-20.0336545736747,-20.6231035244235,
-11.5752365248348));
#72506=CARTESIAN_POINT('Ctrl Pts',(-20.0336312657286,-20.6231216512757,
-11.5752347407489));
#72507=CARTESIAN_POINT('Ctrl Pts',(-20.0336195082778,-20.6231307949786,
-11.5752338407838));
#72508=CARTESIAN_POINT('Ctrl Pts',(-20.0335957815171,-20.6231492467439,
-11.5752320246338));
#72509=CARTESIAN_POINT('Ctrl Pts',(-20.0335838124631,-20.6231585546003,
-11.5752311084686));
#72510=CARTESIAN_POINT('Ctrl Pts',(-20.0335596577322,-20.6231773383556,
-11.5752292595536));
#72511=CARTESIAN_POINT('Ctrl Pts',(-20.0335474723098,-20.6231868140491,
-11.5752283268232));
#72512=CARTESIAN_POINT('Ctrl Pts',(-20.0335228807438,-20.6232059366429,
-11.5752264444642));
#72513=CARTESIAN_POINT('Ctrl Pts',(-20.0335104737562,-20.6232155841916,
-11.5752254947708));
#72514=CARTESIAN_POINT('Ctrl Pts',(-20.0334854335946,-20.623235054722,-11.5752235780672));
#72515=CARTESIAN_POINT('Ctrl Pts',(-20.0334728008742,-20.6232448773427,
-11.5752226110916));
#72516=CARTESIAN_POINT('Ctrl Pts',(-20.0334473043917,-20.6232647017677,
-11.5752206594516));
#72517=CARTESIAN_POINT('Ctrl Pts',(-20.0334344400561,-20.6232747040094,
-11.5752196747433));
#72518=CARTESIAN_POINT('Ctrl Pts',(-20.0334084750853,-20.6232948917387,
-11.5752176872353));
#72519=CARTESIAN_POINT('Ctrl Pts',(-20.0333953743993,-20.623305077257,-11.5752166844316));
#72520=CARTESIAN_POINT('Ctrl Pts',(-20.0333689309668,-20.6233256359919,
-11.5752146602917));
#72521=CARTESIAN_POINT('Ctrl Pts',(-20.0333555884457,-20.6233360090241,
-11.5752136389726));
#72522=CARTESIAN_POINT('Ctrl Pts',(-20.0333286557826,-20.6233569470817,
-11.575211577376));
#72523=CARTESIAN_POINT('Ctrl Pts',(-20.0333150657324,-20.6233675120263,
-11.5752105371055));
#72524=CARTESIAN_POINT('Ctrl Pts',(-20.0332876321185,-20.6233888384608,
-11.5752084371547));
#72525=CARTESIAN_POINT('Ctrl Pts',(-20.033273788974,-20.6233995996148,-11.5752073775064));
#72526=CARTESIAN_POINT('Ctrl Pts',(-20.0304283522789,-20.6256114812766,
-11.5749895680261));
#72527=CARTESIAN_POINT('Ctrl Pts',(-20.0275912314192,-20.627805355082,-11.5747723018109));
#72528=CARTESIAN_POINT('Ctrl Pts',(-20.0210760000583,-20.6328170151961,
-11.5742731672189));
#72529=CARTESIAN_POINT('Ctrl Pts',(-20.0173942073726,-20.6356299403492,
-11.5739909614331));
#72530=CARTESIAN_POINT('Ctrl Pts',(-20.0075614602168,-20.6430912598743,
-11.5732369807269));
#72531=CARTESIAN_POINT('Ctrl Pts',(-20.0013943626232,-20.6477181274058,
-11.5727637624762));
#72532=CARTESIAN_POINT('Ctrl Pts',(-19.9571208653912,-20.6805579018551,
-11.5693650709828));
#72533=CARTESIAN_POINT('Ctrl Pts',(-19.9181043615528,-20.7075150744474,
-11.5663624340112));
#72534=CARTESIAN_POINT('Ctrl Pts',(-19.8739262935959,-20.7358954797653,
-11.5629826349602));
#72535=CARTESIAN_POINT('Ctrl Pts',(-19.8696232086967,-20.7386378941255,
-11.5626536342788));
#72536=CARTESIAN_POINT('Ctrl Pts',(-19.7361460573059,-20.8230276627825,
-11.5524555510168));
#72537=CARTESIAN_POINT('Ctrl Pts',(-19.598519616211,-20.8904659096128,-11.5421895606764));
#72538=CARTESIAN_POINT('Ctrl Pts',(-19.3645534466935,-20.9751928737638,
-11.5260136986025));
#72539=CARTESIAN_POINT('Ctrl Pts',(-19.2721512865808,-21.0017084126554,
-11.5199118666605));
#72540=CARTESIAN_POINT('Ctrl Pts',(-19.1572683192196,-21.0263658600964,
-11.5126938616489));
#72541=CARTESIAN_POINT('Ctrl Pts',(-19.136212364857,-21.0305511921553,-11.5113853579743));
#72542=CARTESIAN_POINT('Ctrl Pts',(-19.1062208018131,-21.0360398455086,
-11.5095413842829));
#72543=CARTESIAN_POINT('Ctrl Pts',(-19.0973354384946,-21.0376072895067,
-11.508997540457));
#72544=CARTESIAN_POINT('Ctrl Pts',(-19.0820037345527,-21.0402109624818,
-11.5080632895427));
#72545=CARTESIAN_POINT('Ctrl Pts',(-19.0755621749183,-21.041274253237,-11.507672027193));
#72546=CARTESIAN_POINT('Ctrl Pts',(-19.0632287999549,-21.0432515257891,
-11.5069252660748));
#72547=CARTESIAN_POINT('Ctrl Pts',(-19.0573378504017,-21.0441704477533,
-11.5065696139974));
#72548=CARTESIAN_POINT('Ctrl Pts',(-19.0420304387359,-21.0464920348363,
-11.5056481048649));
#72549=CARTESIAN_POINT('Ctrl Pts',(-19.032608189996,-21.0478560991988,-11.5050834740262));
#72550=CARTESIAN_POINT('Ctrl Pts',(-19.0005573329577,-21.0522755922057,
-11.5031713655264));
#72551=CARTESIAN_POINT('Ctrl Pts',(-18.9778881304877,-21.0550285339199,
-11.5018334283228));
#72552=CARTESIAN_POINT('Ctrl Pts',(-18.7786169280041,-21.0759623889595,
-11.4901885369016));
#72553=CARTESIAN_POINT('Ctrl Pts',(-18.6004266435321,-21.0722291514489,
-11.4806531542528));
#72554=CARTESIAN_POINT('Ctrl Pts',(-18.340121870918,-21.0337954209121,-11.4663313288045));
#72555=CARTESIAN_POINT('Ctrl Pts',(-18.2563064398102,-21.0161750665568,
-11.4616421432142));
#72556=CARTESIAN_POINT('Ctrl Pts',(-18.1376708697272,-20.9836209664239,
-11.4546156891845));
#72557=CARTESIAN_POINT('Ctrl Pts',(-18.10181905066,-20.9727520979914,-11.4524391971222));
#72558=CARTESIAN_POINT('Ctrl Pts',(-18.0591116052589,-20.9585571681657,
-11.449761417048));
#72559=CARTESIAN_POINT('Ctrl Pts',(-18.0519591543124,-20.9561372945469,
-11.4493100501105));
#72560=CARTESIAN_POINT('Ctrl Pts',(-18.040869774355,-20.9523192104497,-11.448605495434));
#72561=CARTESIAN_POINT('Ctrl Pts',(-18.0369236978897,-20.9509474934926,
-11.4483538484556));
#72562=CARTESIAN_POINT('Ctrl Pts',(-18.0296186535031,-20.9483838864436,
-11.447886213624));
#72563=CARTESIAN_POINT('Ctrl Pts',(-18.0262586256018,-20.9471951908831,
-11.4476704160123));
#72564=CARTESIAN_POINT('Ctrl Pts',(-18.0186762294424,-20.9444911612744,
-11.4471818493433));
#72565=CARTESIAN_POINT('Ctrl Pts',(-18.0144556903384,-20.9429708963362,
-11.4469087911941));
#72566=CARTESIAN_POINT('Ctrl Pts',(-18.0020330502059,-20.938451523183,-11.4461018695659));
#72567=CARTESIAN_POINT('Ctrl Pts',(-17.9938447554281,-20.9354151046728,
-11.4455658617546));
#72568=CARTESIAN_POINT('Ctrl Pts',(-17.9354277464974,-20.9133405459597,
-11.4417134634449));
#72569=CARTESIAN_POINT('Ctrl Pts',(-17.8859251258482,-20.8924490031394,
-11.43829865909));
#72570=CARTESIAN_POINT('Ctrl Pts',(-17.8358135390154,-20.8690166105104,
-11.4347225586648));
#72571=CARTESIAN_POINT('Ctrl Pts',(-17.8343526425792,-20.8683314525241,
-11.4346181983414));
#72572=CARTESIAN_POINT('Ctrl Pts',(-17.6830300437104,-20.7971502314567,
-11.4237973728122));
#72573=CARTESIAN_POINT('Ctrl Pts',(-17.5419538727101,-20.7093133261423,
-11.4126524078956));
#72574=CARTESIAN_POINT('Ctrl Pts',(-17.3481817952745,-20.5544933967912,
-11.3966456620601));
#72575=CARTESIAN_POINT('Ctrl Pts',(-17.2868650396811,-20.4993462430798,
-11.391443369791));
#72576=CARTESIAN_POINT('Ctrl Pts',(-17.2150028042942,-20.4266958213404,
-11.385176868305));
#72577=CARTESIAN_POINT('Ctrl Pts',(-17.2012901825571,-20.4124385996125,
-11.3839725379746));
#72578=CARTESIAN_POINT('Ctrl Pts',(-17.1818158989105,-20.3916144394611,
-11.3822491564036));
#72579=CARTESIAN_POINT('Ctrl Pts',(-17.1758922131555,-20.3852010836314,
-11.3817231495992));
#72580=CARTESIAN_POINT('Ctrl Pts',(-17.1656427958268,-20.373965765426,-11.3808098228625));
#72581=CARTESIAN_POINT('Ctrl Pts',(-17.1612992410656,-20.3691602881184,
-11.3804217477678));
#72582=CARTESIAN_POINT('Ctrl Pts',(-17.1529554953507,-20.3598436080819,
-11.379674258925));
#72583=CARTESIAN_POINT('Ctrl Pts',(-17.1489523912764,-20.3553351095643,
-11.3793147245042));
#72584=CARTESIAN_POINT('Ctrl Pts',(-17.1395029388477,-20.3446006410547,
-11.3784638251503));
#72585=CARTESIAN_POINT('Ctrl Pts',(-17.1340736870449,-20.3383597006392,
-11.377973175));
#72586=CARTESIAN_POINT('Ctrl Pts',(-17.1150155147745,-20.3161912115734,
-11.3762444284302));
#72587=CARTESIAN_POINT('Ctrl Pts',(-17.1015864451089,-20.300092896419,-11.375014545015));
#72588=CARTESIAN_POINT('Ctrl Pts',(-16.9654659817686,-20.131899091542,-11.3624152173509));
#72589=CARTESIAN_POINT('Ctrl Pts',(-16.8641601627928,-19.9637204788182,
-11.3520147333967));
#72590=CARTESIAN_POINT('Ctrl Pts',(-16.7583034625296,-19.7160524409148,
-11.337297523916));
#72591=CARTESIAN_POINT('Ctrl Pts',(-16.7328340676586,-19.6466122475292,
-11.3332149170402));
#72592=CARTESIAN_POINT('Ctrl Pts',(-16.7009389175957,-19.5432092254425,
-11.3270137967667));
#72593=CARTESIAN_POINT('Ctrl Pts',(-16.6916268484878,-19.5101911135058,
-11.3250158591472));
#72594=CARTESIAN_POINT('Ctrl Pts',(-16.6812968559391,-19.4698348678679,
-11.3225361986492));
#72595=CARTESIAN_POINT('Ctrl Pts',(-16.6795093329084,-19.4626968212548,
-11.3220961864667));
#72596=CARTESIAN_POINT('Ctrl Pts',(-16.6767753509654,-19.4515326297265,
-11.3214055676379));
#72597=CARTESIAN_POINT('Ctrl Pts',(-16.6758033953377,-19.447512704823,-11.3211564051586));
#72598=CARTESIAN_POINT('Ctrl Pts',(-16.6740147574145,-19.4400189899952,
-11.320690976177));
#72599=CARTESIAN_POINT('Ctrl Pts',(-16.6731950765745,-19.4365459743117,
-11.3204748846718));
#72600=CARTESIAN_POINT('Ctrl Pts',(-16.671351758678,-19.428646487416,-11.319982509782));
#72601=CARTESIAN_POINT('Ctrl Pts',(-16.6703335920687,-19.4242188023378,
-11.3197059176251));
#72602=CARTESIAN_POINT('Ctrl Pts',(-16.6677291094246,-19.4127234265138,
-11.3189862838825));
#72603=CARTESIAN_POINT('Ctrl Pts',(-16.6661648165223,-19.4056508784201,
-11.3185420286667));
#72604=CARTESIAN_POINT('Ctrl Pts',(-16.6565182475577,-19.3609496466262,
-11.3157253143244));
#72605=CARTESIAN_POINT('Ctrl Pts',(-16.6494276171593,-19.3231169608967,
-11.3133019564691));
#72606=CARTESIAN_POINT('Ctrl Pts',(-16.6413177492058,-19.2722194751253,
-11.310007672671));
#72607=CARTESIAN_POINT('Ctrl Pts',(-16.639382415205,-19.2593055087793,-11.3091689049927));
#72608=CARTESIAN_POINT('Ctrl Pts',(-16.6342012907033,-19.2224073602757,
-11.3067654610224));
#72609=CARTESIAN_POINT('Ctrl Pts',(-16.6312472119723,-19.1983846788938,
-11.3051924166487));
#72610=CARTESIAN_POINT('Ctrl Pts',(-16.6239679875808,-19.1294520813687,
-11.3006636405915));
#72611=CARTESIAN_POINT('Ctrl Pts',(-16.6206657341887,-19.0844478517381,
-11.2976890347353));
#72612=CARTESIAN_POINT('Ctrl Pts',(-16.6142908378506,-18.9301203174101,
-11.2874858142536));
#72613=CARTESIAN_POINT('Ctrl Pts',(-16.6182489877911,-18.8206730275438,
-11.2802556413919));
#72614=CARTESIAN_POINT('Ctrl Pts',(-16.6368877453668,-18.6573127939604,
-11.2696875091259));
#72615=CARTESIAN_POINT('Ctrl Pts',(-16.6452611316731,-18.6028709162452,
-11.2662011542191));
#72616=CARTESIAN_POINT('Ctrl Pts',(-16.6622778449022,-18.5151571175473,
-11.2606474969773));
#72617=CARTESIAN_POINT('Ctrl Pts',(-16.6696241816054,-18.48166279303,-11.2585418233322));
#72618=CARTESIAN_POINT('Ctrl Pts',(-16.6803520144997,-18.4378640974134,
-11.2558065930408));
#72619=CARTESIAN_POINT('Ctrl Pts',(-16.6830032099105,-18.4273878113292,
-11.255153722763));
#72620=CARTESIAN_POINT('Ctrl Pts',(-16.6874778822416,-18.410258551145,-11.2540883859295));
#72621=CARTESIAN_POINT('Ctrl Pts',(-16.689253840375,-18.4035934716542,-11.2536743908326));
#72622=CARTESIAN_POINT('Ctrl Pts',(-16.6927553212726,-18.3907060898778,
-11.2528748939722));
#72623=CARTESIAN_POINT('Ctrl Pts',(-16.694476797333,-18.3844827763128,-11.2524892660685));
#72624=CARTESIAN_POINT('Ctrl Pts',(-16.6985183630847,-18.3701280152444,
-11.2516007649937));
#72625=CARTESIAN_POINT('Ctrl Pts',(-16.7008587623885,-18.3620023627581,
-11.2510985582762));
#72626=CARTESIAN_POINT('Ctrl Pts',(-16.7072862069991,-18.3401793436074,
-11.2497516399945));
#72627=CARTESIAN_POINT('Ctrl Pts',(-16.7114634404168,-18.3265088374717,
-11.2489098719704));
#72628=CARTESIAN_POINT('Ctrl Pts',(-16.7511464134438,-18.2011971691311,
-11.2412094359633));
#72629=CARTESIAN_POINT('Ctrl Pts',(-16.7957251604953,-18.0926344336082,
-11.2346692916207));
#72630=CARTESIAN_POINT('Ctrl Pts',(-16.9236328374399,-17.8424536776135,
-11.2192886908296));
#72631=CARTESIAN_POINT('Ctrl Pts',(-17.0148679750468,-17.7057676535107,
-11.2106344587158));
#72632=CARTESIAN_POINT('Ctrl Pts',(-17.1411812576398,-17.5571540339218,
-11.1994200459266));
#72633=CARTESIAN_POINT('Ctrl Pts',(-17.1619566971105,-17.5337805407049,
-11.1975944553612));
#72634=CARTESIAN_POINT('Ctrl Pts',(-17.1881102377196,-17.5056373174185,
-11.1953064843154));
#72635=CARTESIAN_POINT('Ctrl Pts',(-17.1930060659735,-17.5004222863873,
-11.1948786100337));
#72636=CARTESIAN_POINT('Ctrl Pts',(-17.200743040498,-17.4922641233642,-11.1942029030577));
#72637=CARTESIAN_POINT('Ctrl Pts',(-17.2035665008124,-17.4893041883865,
-11.1939564142953));
#72638=CARTESIAN_POINT('Ctrl Pts',(-17.2088734410351,-17.4837729199301,
-11.1934932566674));
#72639=CARTESIAN_POINT('Ctrl Pts',(-17.2113548610946,-17.4811996873116,
-11.1932767460596));
#72640=CARTESIAN_POINT('Ctrl Pts',(-17.2170517747477,-17.4753218557642,
-11.1927798054227));
#72641=CARTESIAN_POINT('Ctrl Pts',(-17.2202715451111,-17.4720214786387,
-11.192499043489));
#72642=CARTESIAN_POINT('Ctrl Pts',(-17.2302634605219,-17.461846132948,-11.1916281338745));
#72643=CARTESIAN_POINT('Ctrl Pts',(-17.2370717411971,-17.4550070449214,
-11.1910352497287));
#72644=CARTESIAN_POINT('Ctrl Pts',(-17.307521700781,-17.3851994474055,-11.1849080563275));
#72645=CARTESIAN_POINT('Ctrl Pts',(-17.3750433680705,-17.3262886361878,
-11.1791036289618));
#72646=CARTESIAN_POINT('Ctrl Pts',(-17.4930927077582,-17.235798732497,-11.1693288862232));
#72647=CARTESIAN_POINT('Ctrl Pts',(-17.54159556474,-17.2017516551551,-11.1654055534536));
#72648=CARTESIAN_POINT('Ctrl Pts',(-17.7187164040156,-17.0882035412027,
-11.1515189926062));
#72649=CARTESIAN_POINT('Ctrl Pts',(-17.8543634099491,-17.0204738700821,
-11.1417108762248));
#72650=CARTESIAN_POINT('Ctrl Pts',(-18.0159927270331,-16.9603661461655,
-11.131120101357));
#72651=CARTESIAN_POINT('Ctrl Pts',(-18.0360051205492,-16.9532646369299,
-11.1298259899217));
#72652=CARTESIAN_POINT('Ctrl Pts',(-18.0646315724498,-16.9435887865455,
-11.1279986095254));
#72653=CARTESIAN_POINT('Ctrl Pts',(-18.0731599095603,-16.9407665294933,
-11.1274571701216));
#72654=CARTESIAN_POINT('Ctrl Pts',(-18.0879102482788,-16.9359891958493,
-11.1265257547475));
#72655=CARTESIAN_POINT('Ctrl Pts',(-18.0941237452958,-16.9340084465304,
-11.1261349371457));
#72656=CARTESIAN_POINT('Ctrl Pts',(-18.1060429328967,-16.9302694130194,
-11.1253881432459));
#72657=CARTESIAN_POINT('Ctrl Pts',(-18.1117470936753,-16.9285064946601,
-11.1250320178821));
#72658=CARTESIAN_POINT('Ctrl Pts',(-18.1266094453857,-16.9239819499955,
-11.1241073753115));
#72659=CARTESIAN_POINT('Ctrl Pts',(-18.1357790966937,-16.9212582014469,
-11.1235401012597));
#72660=CARTESIAN_POINT('Ctrl Pts',(-18.1671627411517,-16.9121670380822,
-11.1216092456665));
#72661=CARTESIAN_POINT('Ctrl Pts',(-18.1894628661008,-16.9061010870061,
-11.1202554648303));
#72662=CARTESIAN_POINT('Ctrl Pts',(-18.3803334569641,-16.8575236264456,
-11.1088120330079));
#72663=CARTESIAN_POINT('Ctrl Pts',(-18.5534464133171,-16.8355599523234,
-11.099457032121));
#72664=CARTESIAN_POINT('Ctrl Pts',(-18.815462624508,-16.8347320222064,-11.0852040104298));
#72665=CARTESIAN_POINT('Ctrl Pts',(-18.9035392322254,-16.8399597932138,
-11.0803815958537));
#72666=CARTESIAN_POINT('Ctrl Pts',(-19.028856184673,-16.8552879573845,-11.0731754996182));
#72667=CARTESIAN_POINT('Ctrl Pts',(-19.0665522244061,-16.8609356371533,
-11.0709621361512));
#72668=CARTESIAN_POINT('Ctrl Pts',(-19.1115438729607,-16.8689236202211,
-11.068243488057));
#72669=CARTESIAN_POINT('Ctrl Pts',(-19.1190078669846,-16.8702902415531,
-11.0677899153578));
#72670=CARTESIAN_POINT('Ctrl Pts',(-19.1305775019918,-16.8724729369049,
-11.0670826552624));
#72671=CARTESIAN_POINT('Ctrl Pts',(-19.1346884285145,-16.8732611265988,
-11.066830527709));
#72672=CARTESIAN_POINT('Ctrl Pts',(-19.1422946906124,-16.8747428796379,
-11.0663624566346));
#72673=CARTESIAN_POINT('Ctrl Pts',(-19.145790622846,-16.8754330781707,-11.0661467062739));
#72674=CARTESIAN_POINT('Ctrl Pts',(-19.1536733537035,-16.8770100466767,
-11.0656588326937));
#72675=CARTESIAN_POINT('Ctrl Pts',(-19.1580590667994,-16.8779018978805,
-11.0653864240091));
#72676=CARTESIAN_POINT('Ctrl Pts',(-19.1693179224785,-16.8802286309406,
-11.0646846693478));
#72677=CARTESIAN_POINT('Ctrl Pts',(-19.176186751448,-16.8816837987949,-11.0642542054727));
#72678=CARTESIAN_POINT('Ctrl Pts',(-19.2171490559425,-16.8905748495753,
-11.0616736947725));
#72679=CARTESIAN_POINT('Ctrl Pts',(-19.251059575373,-16.8988181446468,-11.0594818296684));
#72680=CARTESIAN_POINT('Ctrl Pts',(-19.3010310369819,-16.9122820858429,
-11.0561842401516));
#72681=CARTESIAN_POINT('Ctrl Pts',(-19.3172601511958,-16.9168634114519,
-11.0551025635541));
#72682=CARTESIAN_POINT('Ctrl Pts',(-19.3343465824947,-16.9219079110824,
-11.0539535345151));
#72683=CARTESIAN_POINT('Ctrl Pts',(-19.3352605937441,-16.9221784297616,
-11.0538920380399));
#72684=CARTESIAN_POINT('Ctrl Pts',(-19.3406451319327,-16.9237760403013,
-11.053529574103));
#72685=CARTESIAN_POINT('Ctrl Pts',(-19.3451114216255,-16.9251172760521,
-11.0532281848643));
#72686=CARTESIAN_POINT('Ctrl Pts',(-19.3733200192054,-16.9336900866297,
-11.0513201154294));
#72687=CARTESIAN_POINT('Ctrl Pts',(-19.3969374990588,-16.9413237942379,
-11.0497023113939));
#72688=CARTESIAN_POINT('Ctrl Pts',(-19.4575335737938,-16.9620935078351,
-11.0455070938697));
#72689=CARTESIAN_POINT('Ctrl Pts',(-19.4942909164965,-16.9758455796272,
-11.0429191744637));
#72690=CARTESIAN_POINT('Ctrl Pts',(-19.6319039644652,-17.0317389395767,
-11.0331074510814));
#72691=CARTESIAN_POINT('Ctrl Pts',(-19.7298347048603,-17.0806500117974,
-11.0258811083959));
#72692=CARTESIAN_POINT('Ctrl Pts',(-19.8707066089787,-17.1652119787485,
-11.0153210185736));
#72693=CARTESIAN_POINT('Ctrl Pts',(-19.9167399781432,-17.1953439982526,
-11.0118388494714));
#72694=CARTESIAN_POINT('Ctrl Pts',(-19.9894591958985,-17.2470998201683,
-11.0062910797199));
#72695=CARTESIAN_POINT('Ctrl Pts',(-20.0168825433592,-17.2676380997185,
-11.0041872091145));
#72696=CARTESIAN_POINT('Ctrl Pts',(-20.0522837211303,-17.2955176627458,
-11.0014539428101));
#72697=CARTESIAN_POINT('Ctrl Pts',(-20.0607195885365,-17.3022664326622,
-11.0008012753337));
#72698=CARTESIAN_POINT('Ctrl Pts',(-20.0744558861512,-17.3134291034181,
-10.9997361845875));
#72699=CARTESIAN_POINT('Ctrl Pts',(-20.0797869824924,-17.3178047958252,
-10.9993222341393));
#72700=CARTESIAN_POINT('Ctrl Pts',(-20.0900678100271,-17.3263275882316,
-10.9985227648716));
#72701=CARTESIAN_POINT('Ctrl Pts',(-20.0950201309793,-17.3304714309419,
-10.9981371202192));
#72702=CARTESIAN_POINT('Ctrl Pts',(-20.1064149699957,-17.3400950147911,
-10.9972484967315));
#72703=CARTESIAN_POINT('Ctrl Pts',(-20.1128437920656,-17.3455908580134,
-10.9967461849391));
#72704=CARTESIAN_POINT('Ctrl Pts',(-20.1300532705622,-17.3604822473122,
-10.995398798728));
#72705=CARTESIAN_POINT('Ctrl Pts',(-20.1407720675095,-17.369948845206,-10.9945566710879));
#72706=CARTESIAN_POINT('Ctrl Pts',(-20.2387839507698,-17.4582945132311,
-10.9868265981097));
#72707=CARTESIAN_POINT('Ctrl Pts',(-20.3194606300363,-17.5442177894591,
-10.9802601224696));
#72708=CARTESIAN_POINT('Ctrl Pts',(-20.4942609928979,-17.7645918866182,
-10.9648656021939));
#72709=CARTESIAN_POINT('Ctrl Pts',(-20.5807193416625,-17.9041106389875,
-10.9562205072344));
#72710=CARTESIAN_POINT('Ctrl Pts',(-20.6634192119356,-18.0802252846467,
-10.9450299844428));
#72711=CARTESIAN_POINT('Ctrl Pts',(-20.6759748602771,-18.1085647248755,
-10.9432200940925));
#72712=CARTESIAN_POINT('Ctrl Pts',(-20.690648753618,-18.143751561138,-10.9409496141373));
#72713=CARTESIAN_POINT('Ctrl Pts',(-20.6933610185081,-18.1503490286847,
-10.9405229093265));
#72714=CARTESIAN_POINT('Ctrl Pts',(-20.6975744493935,-18.1607471457256,
-10.9398486397909));
#72715=CARTESIAN_POINT('Ctrl Pts',(-20.6990980709941,-18.1645387194061,
-10.9396024095043));
#72716=CARTESIAN_POINT('Ctrl Pts',(-20.7019342811252,-18.1716561977018,
-10.9391394652371));
#72717=CARTESIAN_POINT('Ctrl Pts',(-20.703249424435,-18.1749810244938,-10.9389229078748));
#72718=CARTESIAN_POINT('Ctrl Pts',(-20.7062437525257,-18.1826074448077,
-10.9384254974222));
#72719=CARTESIAN_POINT('Ctrl Pts',(-20.7079172852275,-18.1869111989385,
-10.9381443100713));
#72720=CARTESIAN_POINT('Ctrl Pts',(-20.7130574314315,-18.2002590231849,
-10.937270793411));
#72721=CARTESIAN_POINT('Ctrl Pts',(-20.7164760103375,-18.2093212852235,
-10.9366757044127));
#72722=CARTESIAN_POINT('Ctrl Pts',(-20.7565245106005,-18.3177322788394,
-10.9295352707546));
#72723=CARTESIAN_POINT('Ctrl Pts',(-20.7857089113694,-18.4196597363177,
-10.9226145016515));
#72724=CARTESIAN_POINT('Ctrl Pts',(-20.8362075107609,-18.6638812322754,
-10.9061648035184));
#72725=CARTESIAN_POINT('Ctrl Pts',(-20.8509047688548,-18.8070440802342,
-10.8966462024059));
#72726=CARTESIAN_POINT('Ctrl Pts',(-20.8510404642358,-19.0125966095008,
-10.8835935804314));
#72727=CARTESIAN_POINT('Ctrl Pts',(-20.8483582573966,-19.074567055652,-10.8797325381029));
#72728=CARTESIAN_POINT('Ctrl Pts',(-20.8418780036544,-19.1487067130386,
-10.875199750235));
#72729=CARTESIAN_POINT('Ctrl Pts',(-20.8406878626907,-19.16106809596,-10.8744468386955));
#72730=CARTESIAN_POINT('Ctrl Pts',(-20.8385539133339,-19.1813590539228,
-10.8732154675641));
#72731=CARTESIAN_POINT('Ctrl Pts',(-20.8376739010711,-19.1892949018066,
-10.872735012191));
#72732=CARTESIAN_POINT('Ctrl Pts',(-20.8360103029197,-19.2035598415205,
-10.8718733679328));
#72733=CARTESIAN_POINT('Ctrl Pts',(-20.8352429788777,-19.2098906988285,
-10.8714916715242));
#72734=CARTESIAN_POINT('Ctrl Pts',(-20.8335469916007,-19.2233732429876,
-10.8706802559566));
#72735=CARTESIAN_POINT('Ctrl Pts',(-20.8326103659402,-19.2305238605445,
-10.8702507931481));
#72736=CARTESIAN_POINT('Ctrl Pts',(-20.8299874451884,-19.2497836479508,
-10.8690963550652));
#72737=CARTESIAN_POINT('Ctrl Pts',(-20.8282327461388,-19.2618833422834,
-10.8683735464714));
#72738=CARTESIAN_POINT('Ctrl Pts',(-20.8189028622638,-19.3225155765967,
-10.8647630127091));
#72739=CARTESIAN_POINT('Ctrl Pts',(-20.8097446709085,-19.3707915360266,
-10.8619258064585));
#72740=CARTESIAN_POINT('Ctrl Pts',(-20.7790242589775,-19.5067116634044,
-10.8540036864043));
#72741=CARTESIAN_POINT('Ctrl Pts',(-20.7535279435943,-19.5933555926682,
-10.8490364150279));
#72742=CARTESIAN_POINT('Ctrl Pts',(-20.7225805823871,-19.6781103685755,
-10.8441190550425));
#72743=CARTESIAN_POINT('Origin',(-18.734,-18.952,0.));
#72744=CARTESIAN_POINT('',(-20.722580582123,-19.6781103692989,-10.0464611886058));
#72745=CARTESIAN_POINT('',(-20.7219729237028,-19.6778789621695,-10.2662522608197));
#72746=CARTESIAN_POINT('',(-20.7225805821191,-19.6781103693095,0.));
#72747=CARTESIAN_POINT('',(-20.8538228835136,-18.9530774369207,-10.3109437209775));
#72748=CARTESIAN_POINT('Ctrl Pts',(-20.7219729237027,-19.6778789621698,
-10.2662522608197));
#72749=CARTESIAN_POINT('Ctrl Pts',(-20.787539735307,-19.5036327148231,-10.2774434356492));
#72750=CARTESIAN_POINT('Ctrl Pts',(-20.8444160839083,-19.2611105174517,
-10.2923405890351));
#72751=CARTESIAN_POINT('Ctrl Pts',(-20.8542039878978,-19.0144660717244,
-10.307237742421));
#72752=CARTESIAN_POINT('Ctrl Pts',(-20.8538228835136,-18.9530774369207,
-10.3109437209775));
#72753=CARTESIAN_POINT('Ctrl Pts',(-20.8509997772493,-18.9529711470399,
-10.3093226856846));
#72754=CARTESIAN_POINT('Ctrl Pts',(-20.8510794193682,-18.7793595916912,
-10.3204900561849));
#72755=CARTESIAN_POINT('Ctrl Pts',(-20.8298038944403,-18.6063867465604,
-10.3322030597167));
#72756=CARTESIAN_POINT('Ctrl Pts',(-20.7727769716693,-18.3785693060707,
-10.3473694074294));
#72757=CARTESIAN_POINT('Ctrl Pts',(-20.7553480080759,-18.3198705581746,
-10.3512605836352));
#72758=CARTESIAN_POINT('Ctrl Pts',(-20.7233403127886,-18.2270290779853,
-10.3573784312497));
#72759=CARTESIAN_POINT('Ctrl Pts',(-20.7103668064488,-18.1923736213319,
-10.3596539082093));
#72760=CARTESIAN_POINT('Ctrl Pts',(-20.6923256027683,-18.1477778926987,
-10.3625732349727));
#72761=CARTESIAN_POINT('Ctrl Pts',(-20.6880792039238,-18.1375143730626,
-10.363244502009));
#72762=CARTESIAN_POINT('Ctrl Pts',(-20.6810393040183,-18.1208709831831,
-10.3643321719418));
#72763=CARTESIAN_POINT('Ctrl Pts',(-20.6782947910262,-18.1144707399865,
-10.364750228847));
#72764=CARTESIAN_POINT('Ctrl Pts',(-20.6729543848587,-18.1021845649081,
-10.3655523895481));
#72765=CARTESIAN_POINT('Ctrl Pts',(-20.6703631503778,-18.0962967035517,
-10.3659366467752));
#72766=CARTESIAN_POINT('Ctrl Pts',(-20.6643661714385,-18.082836969157,-10.366814742967));
#72767=CARTESIAN_POINT('Ctrl Pts',(-20.6609426267439,-18.0752731062338,
-10.3673079656299));
#72768=CARTESIAN_POINT('Ctrl Pts',(-20.6517237262486,-18.055220055506,-10.3686150802324));
#72769=CARTESIAN_POINT('Ctrl Pts',(-20.6458508213901,-18.0427668015452,
-10.3694262976481));
#72770=CARTESIAN_POINT('Ctrl Pts',(-20.5997890217786,-17.9475145479618,
-10.3756289861628));
#72771=CARTESIAN_POINT('Ctrl Pts',(-20.5543581860886,-17.8673531545177,
-10.3808303029813));
#72772=CARTESIAN_POINT('Ctrl Pts',(-20.4266263404313,-17.6727378440846,
-10.3937058489615));
#72773=CARTESIAN_POINT('Ctrl Pts',(-20.3378682033472,-17.5630795093536,
-10.4011868368574));
#72774=CARTESIAN_POINT('Ctrl Pts',(-20.2015575085882,-17.425310348179,-10.4119104618055));
#72775=CARTESIAN_POINT('Ctrl Pts',(-20.162822177308,-17.3889988003595,-10.414890161463));
#72776=CARTESIAN_POINT('Ctrl Pts',(-20.1088699145807,-17.3421053719128,
-10.4190171484939));
#72777=CARTESIAN_POINT('Ctrl Pts',(-20.0948169897376,-17.3302093016445,
-10.4200901189935));
#72778=CARTESIAN_POINT('Ctrl Pts',(-20.0738350991701,-17.3129124410464,
-10.4216922816779));
#72779=CARTESIAN_POINT('Ctrl Pts',(-20.0670244445388,-17.3073687515419,
-10.4222123618597));
#72780=CARTESIAN_POINT('Ctrl Pts',(-20.054694019646,-17.2974590259749,-10.423154393972));
#72781=CARTESIAN_POINT('Ctrl Pts',(-20.0491865537469,-17.2930778035314,
-10.4235753175168));
#72782=CARTESIAN_POINT('Ctrl Pts',(-20.040459814539,-17.2862064002273,-10.4242427154831));
#72783=CARTESIAN_POINT('Ctrl Pts',(-20.0372549728867,-17.2836978573849,
-10.4244879045828));
#72784=CARTESIAN_POINT('Ctrl Pts',(-20.0340336348583,-17.2811913489641,
-10.4247344695675));
#72785=CARTESIAN_POINT('Ctrl Pts',(-20.0340243211539,-17.2811841021382,
-10.4247351824503));
#72786=CARTESIAN_POINT('Ctrl Pts',(-20.0340056579227,-17.2811695808643,
-10.4247366109597));
#72787=CARTESIAN_POINT('Ctrl Pts',(-20.033996308311,-17.2811623063511,-10.4247373265928));
#72788=CARTESIAN_POINT('Ctrl Pts',(-20.0339775732599,-17.2811477297012,
-10.4247387606032));
#72789=CARTESIAN_POINT('Ctrl Pts',(-20.0339681873699,-17.2811404272149,
-10.4247394790151));
#72790=CARTESIAN_POINT('Ctrl Pts',(-20.0339493787154,-17.2811257938074,
-10.4247409186631));
#72791=CARTESIAN_POINT('Ctrl Pts',(-20.0339399567985,-17.2811184635465,
-10.4247416398344));
#72792=CARTESIAN_POINT('Ctrl Pts',(-20.03392107619,-17.2811037746705,-10.4247430849939));
#72793=CARTESIAN_POINT('Ctrl Pts',(-20.0339116170876,-17.2810964157366,
-10.4247438090134));
#72794=CARTESIAN_POINT('Ctrl Pts',(-20.033891928788,-17.2810810990237,-10.4247453159992));
#72795=CARTESIAN_POINT('Ctrl Pts',(-20.0338816997124,-17.2810731413611,
-10.4247460989564));
#72796=CARTESIAN_POINT('Ctrl Pts',(-20.0338610630875,-17.2810570874973,
-10.4247476785337));
#72797=CARTESIAN_POINT('Ctrl Pts',(-20.0338506553949,-17.28104899119,-10.424748475165));
#72798=CARTESIAN_POINT('Ctrl Pts',(-20.0338296579193,-17.2810326572391,
-10.4247500823675));
#72799=CARTESIAN_POINT('Ctrl Pts',(-20.0338190678582,-17.2810244193848,
-10.4247508929602));
#72800=CARTESIAN_POINT('Ctrl Pts',(-20.0337977012581,-17.2810077989438,
-10.4247525284215));
#72801=CARTESIAN_POINT('Ctrl Pts',(-20.0337869252412,-17.280999416769,-10.4247533532503));
#72802=CARTESIAN_POINT('Ctrl Pts',(-20.0337651829476,-17.2809825047624,
-10.4247550174734));
#72803=CARTESIAN_POINT('Ctrl Pts',(-20.0337542164602,-17.2809739747727,
-10.424755856884));
#72804=CARTESIAN_POINT('Ctrl Pts',(-20.0337320891588,-17.2809567639912,
-10.4247575505822));
#72805=CARTESIAN_POINT('Ctrl Pts',(-20.0337209284337,-17.2809480832747,
-10.4247584048631));
#72806=CARTESIAN_POINT('Ctrl Pts',(-20.0336984085359,-17.280930567853,-10.4247601286175));
#72807=CARTESIAN_POINT('Ctrl Pts',(-20.0336870491494,-17.2809217329879,
-10.4247609981075));
#72808=CARTESIAN_POINT('Ctrl Pts',(-20.0336641275913,-17.2809039059147,
-10.4247627526122));
#72809=CARTESIAN_POINT('Ctrl Pts',(-20.0336525653564,-17.2808949136643,
-10.4247636376319));
#72810=CARTESIAN_POINT('Ctrl Pts',(-20.0336292333611,-17.2808767681539,
-10.424765423559));
#72811=CARTESIAN_POINT('Ctrl Pts',(-20.0336174638869,-17.2808676151237,
-10.4247663244446));
#72812=CARTESIAN_POINT('Ctrl Pts',(-20.0335937128453,-17.2808491445224,
-10.4247681424534));
#72813=CARTESIAN_POINT('Ctrl Pts',(-20.0335817313709,-17.2808398270312,
-10.4247690595696));
#72814=CARTESIAN_POINT('Ctrl Pts',(-20.0308946390714,-17.2787502341517,
-10.4249747421063));
#72815=CARTESIAN_POINT('Ctrl Pts',(-20.0282145952773,-17.2766764298895,
-10.4251799677509));
#72816=CARTESIAN_POINT('Ctrl Pts',(-20.0219399979129,-17.2718452196714,
-10.4256606326095));
#72817=CARTESIAN_POINT('Ctrl Pts',(-20.0183415796849,-17.2690929229766,
-10.4259364266806));
#72818=CARTESIAN_POINT('Ctrl Pts',(-20.0073758593416,-17.2607613038662,
-10.4267772194265));
#72819=CARTESIAN_POINT('Ctrl Pts',(-19.999980946506,-17.2552187405541,-10.4273446934099));
#72820=CARTESIAN_POINT('Ctrl Pts',(-19.9401409584356,-17.2109769932916,
-10.4319388993246));
#72821=CARTESIAN_POINT('Ctrl Pts',(-19.8859754012468,-17.174673903762,-10.4361100043851));
#72822=CARTESIAN_POINT('Ctrl Pts',(-19.7079132361217,-17.0668940801398,
-10.4496551322327));
#72823=CARTESIAN_POINT('Ctrl Pts',(-19.5784113480963,-17.0054378217447,
-10.4592335235597));
#72824=CARTESIAN_POINT('Ctrl Pts',(-19.3473606168183,-16.9232236623335,
-10.4751490732572));
#72825=CARTESIAN_POINT('Ctrl Pts',(-19.2486572182595,-16.8959654732595,
-10.4816192969437));
#72826=CARTESIAN_POINT('Ctrl Pts',(-19.1338549727237,-16.873052269362,-10.4887581511366));
#72827=CARTESIAN_POINT('Ctrl Pts',(-19.1193234232712,-16.8703099311315,
-10.4896550406672));
#72828=CARTESIAN_POINT('Ctrl Pts',(-19.097119593072,-16.8663601826252,-10.4910154555303));
#72829=CARTESIAN_POINT('Ctrl Pts',(-19.0894676473943,-16.8650423960097,
-10.4914824805236));
#72830=CARTESIAN_POINT('Ctrl Pts',(-19.0755338120865,-16.8627216270455,
-10.492329684243));
#72831=CARTESIAN_POINT('Ctrl Pts',(-19.0692543488453,-16.8617048085398,
-10.4927102982376));
#72832=CARTESIAN_POINT('Ctrl Pts',(-19.0556888634034,-16.8595708836126,
-10.4935300100819));
#72833=CARTESIAN_POINT('Ctrl Pts',(-19.04840138055,-16.8584634930436,-10.4939687954227));
#72834=CARTESIAN_POINT('Ctrl Pts',(-19.0286282160052,-16.8555643791738,
-10.4951551855948));
#72835=CARTESIAN_POINT('Ctrl Pts',(-19.016131939635,-16.8538461264881,-10.495900462443));
#72836=CARTESIAN_POINT('Ctrl Pts',(-18.955303979036,-16.8460354798875,-10.4995072602386));
#72837=CARTESIAN_POINT('Ctrl Pts',(-18.906784966137,-16.8415005559573,-10.5023194526611));
#72838=CARTESIAN_POINT('Ctrl Pts',(-18.8174408792678,-16.8362520116136,
-10.5074055673432));
#72839=CARTESIAN_POINT('Ctrl Pts',(-18.7766700749188,-16.8350372132828,
-10.5096915279946));
#72840=CARTESIAN_POINT('Ctrl Pts',(-18.6015149717955,-16.8348810016189,
-10.5194116910763));
#72841=CARTESIAN_POINT('Ctrl Pts',(-18.4674400710306,-16.8475546496889,
-10.5265773662841));
#72842=CARTESIAN_POINT('Ctrl Pts',(-18.2739305793158,-16.8846462265019,
-10.5374062461092));
#72843=CARTESIAN_POINT('Ctrl Pts',(-18.2129475501003,-16.8991681280966,
-10.5408963489381));
#72844=CARTESIAN_POINT('Ctrl Pts',(-18.122979145102,-16.9248596307359,-10.5462782755912));
#72845=CARTESIAN_POINT('Ctrl Pts',(-18.0934463843998,-16.9339971752689,
-10.5480834842668));
#72846=CARTESIAN_POINT('Ctrl Pts',(-18.0573649175315,-16.9460327110222,
-10.5503487474621));
#72847=CARTESIAN_POINT('Ctrl Pts',(-18.0506153222674,-16.9483220872038,
-10.5507751013617));
#72848=CARTESIAN_POINT('Ctrl Pts',(-18.0400157032895,-16.9519771294003,
-10.551448939555));
#72849=CARTESIAN_POINT('Ctrl Pts',(-18.0361577805577,-16.9533199547908,
-10.5516950922531));
#72850=CARTESIAN_POINT('Ctrl Pts',(-18.0289301690009,-16.9558591433505,
-10.552157972696));
#72851=CARTESIAN_POINT('Ctrl Pts',(-18.0255596165151,-16.9570528807664,
-10.5523745443152));
#72852=CARTESIAN_POINT('Ctrl Pts',(-18.0178412860028,-16.9598084833635,
-10.5528720968145));
#72853=CARTESIAN_POINT('Ctrl Pts',(-18.013495597809,-16.9613760405134,-10.5531534126666));
#72854=CARTESIAN_POINT('Ctrl Pts',(-18.0000447644388,-16.9662777804661,
-10.5540277177136));
#72855=CARTESIAN_POINT('Ctrl Pts',(-17.9909575203233,-16.9696602495671,
-10.5546234736399));
#72856=CARTESIAN_POINT('Ctrl Pts',(-17.8885299935141,-17.0085892236044,
-10.5613935871788));
#72857=CARTESIAN_POINT('Ctrl Pts',(-17.7978047603853,-17.0506324095215,
-10.567902760316));
#72858=CARTESIAN_POINT('Ctrl Pts',(-17.6933381517651,-17.1083374168986,
-10.5757659955355));
#72859=CARTESIAN_POINT('Ctrl Pts',(-17.6764101759332,-17.1179954858049,
-10.5770525672602));
#72860=CARTESIAN_POINT('Ctrl Pts',(-17.565739975038,-17.1831789414606,-10.5855376920495));
#72861=CARTESIAN_POINT('Ctrl Pts',(-17.4762631147445,-17.2456410613889,
-10.5927393033561));
#72862=CARTESIAN_POINT('Ctrl Pts',(-17.333975943132,-17.3622679320992,-10.6045598990233));
#72863=CARTESIAN_POINT('Ctrl Pts',(-17.2785272354868,-17.4128714857016,
-10.6092790984574));
#72864=CARTESIAN_POINT('Ctrl Pts',(-17.2126800076809,-17.4797133151403,
-10.615027018531));
#72865=CARTESIAN_POINT('Ctrl Pts',(-17.1996621532909,-17.4932848086699,
-10.6161711480857));
#72866=CARTESIAN_POINT('Ctrl Pts',(-17.1809881198082,-17.5132796428476,
-10.6178243089738));
#72867=CARTESIAN_POINT('Ctrl Pts',(-17.1751876009825,-17.5195663805517,
-10.6183395332425));
#72868=CARTESIAN_POINT('Ctrl Pts',(-17.1650808492612,-17.530654408848,-10.6192403576289));
#72869=CARTESIAN_POINT('Ctrl Pts',(-17.1607581863951,-17.5354405101109,
-10.6196266534362));
#72870=CARTESIAN_POINT('Ctrl Pts',(-17.1524043866532,-17.5447753360454,
-10.6203752060694));
#72871=CARTESIAN_POINT('Ctrl Pts',(-17.1483708394203,-17.5493218097851,
-10.6207375623374));
#72872=CARTESIAN_POINT('Ctrl Pts',(-17.1387709985879,-17.5602367399885,
-10.6216022347255));
#72873=CARTESIAN_POINT('Ctrl Pts',(-17.1332231541187,-17.5666213399545,
-10.6221037800799));
#72874=CARTESIAN_POINT('Ctrl Pts',(-17.1133174192485,-17.5898085889461,
-10.6239102185812));
#72875=CARTESIAN_POINT('Ctrl Pts',(-17.099184289931,-17.6068029451931,-10.6252058828932));
#72876=CARTESIAN_POINT('Ctrl Pts',(-16.9688591091537,-17.7686005169474,
-10.637289142984));
#72877=CARTESIAN_POINT('Ctrl Pts',(-16.8719253322914,-17.9278707889274,
-10.6472193997445));
#72878=CARTESIAN_POINT('Ctrl Pts',(-16.7646839404573,-18.1710399562158,
-10.6617076839513));
#72879=CARTESIAN_POINT('Ctrl Pts',(-16.7365514954819,-18.246095048847,-10.6661125560944));
#72880=CARTESIAN_POINT('Ctrl Pts',(-16.7020314371913,-18.3569453537787,
-10.6727537259724));
#72881=CARTESIAN_POINT('Ctrl Pts',(-16.6922024433507,-18.3915995524339,
-10.6748487593431));
#72882=CARTESIAN_POINT('Ctrl Pts',(-16.6814095747168,-18.4337169889009,
-10.6774362028975));
#72883=CARTESIAN_POINT('Ctrl Pts',(-16.679594672032,-18.4409584378852,-10.6778825324453));
#72884=CARTESIAN_POINT('Ctrl Pts',(-16.6768283685089,-18.4522488847521,
-10.678580906465));
#72885=CARTESIAN_POINT('Ctrl Pts',(-16.6758505138807,-18.4562914256275,
-10.6788314533667));
#72886=CARTESIAN_POINT('Ctrl Pts',(-16.6740564191552,-18.463805203277,-10.6792981009882));
#72887=CARTESIAN_POINT('Ctrl Pts',(-16.6732370343696,-18.4672756301861,
-10.679514018183));
#72888=CARTESIAN_POINT('Ctrl Pts',(-16.6714010003066,-18.475140782277,-10.6800042231805));
#72889=CARTESIAN_POINT('Ctrl Pts',(-16.670389631716,-18.4795366743295,-10.6802788085906));
#72890=CARTESIAN_POINT('Ctrl Pts',(-16.6678144193574,-18.4908958046621,
-10.6809898501807));
#72891=CARTESIAN_POINT('Ctrl Pts',(-16.6662717386905,-18.4978637135345,
-10.6814274735406));
#72892=CARTESIAN_POINT('Ctrl Pts',(-16.6570111496377,-18.5407170673958,
-10.6841272778506));
#72893=CARTESIAN_POINT('Ctrl Pts',(-16.6501929059821,-18.5767881192622,
-10.6864357473103));
#72894=CARTESIAN_POINT('Ctrl Pts',(-16.616998226469,-18.7814180918168,-10.6996659054849));
#72895=CARTESIAN_POINT('Ctrl Pts',(-16.6101361683581,-18.9525036638496,
-10.7111777637828));
#72896=CARTESIAN_POINT('Ctrl Pts',(-16.6315580065215,-19.2175250193883,
-10.7284557937702));
#72897=CARTESIAN_POINT('Ctrl Pts',(-16.6456362937023,-19.3118710039997,
-10.7345086108143));
#72898=CARTESIAN_POINT('Ctrl Pts',(-16.6705999748074,-19.4258421294952,
-10.7416752218674));
#72899=CARTESIAN_POINT('Ctrl Pts',(-16.6754903028518,-19.446655341638,-10.7429782936529));
#72900=CARTESIAN_POINT('Ctrl Pts',(-16.6828881243915,-19.4761280468211,
-10.7448160072132));
#72901=CARTESIAN_POINT('Ctrl Pts',(-16.685136805431,-19.4848505884275,-10.7453589457638));
#72902=CARTESIAN_POINT('Ctrl Pts',(-16.689110543327,-19.4998674089627,-10.7462921285862));
#72903=CARTESIAN_POINT('Ctrl Pts',(-16.6908091466947,-19.5061684998858,
-10.7466832229823));
#72904=CARTESIAN_POINT('Ctrl Pts',(-16.6941161130725,-19.518214015266,-10.7474299942396));
#72905=CARTESIAN_POINT('Ctrl Pts',(-16.6957196698045,-19.5239596837978,
-10.7477858228173));
#72906=CARTESIAN_POINT('Ctrl Pts',(-16.6999500459863,-19.538873701343,-10.7487085025316));
#72907=CARTESIAN_POINT('Ctrl Pts',(-16.7026145921048,-19.548031279268,-10.7492741211305));
#72908=CARTESIAN_POINT('Ctrl Pts',(-16.7118975924196,-19.5791498444912,
-10.7511932387757));
#72909=CARTESIAN_POINT('Ctrl Pts',(-16.7188111594146,-19.6010216263463,
-10.7525371004372));
#72910=CARTESIAN_POINT('Ctrl Pts',(-16.7819128938809,-19.7899118602451,
-10.7641101260313));
#72911=CARTESIAN_POINT('Ctrl Pts',(-16.85839321266,-19.9494197709131,-10.7735810672016));
#72912=CARTESIAN_POINT('Ctrl Pts',(-17.0005664995918,-20.1703504946566,
-10.7878777857968));
#72913=CARTESIAN_POINT('Ctrl Pts',(-17.0517807733767,-20.2401404179923,
-10.7926143204675));
#72914=CARTESIAN_POINT('Ctrl Pts',(-17.1312328492206,-20.3355632306599,
-10.7997046831101));
#72915=CARTESIAN_POINT('Ctrl Pts',(-17.1561189047737,-20.3638783966051,
-10.8018943724424));
#72916=CARTESIAN_POINT('Ctrl Pts',(-17.1868891626435,-20.3970585714183,
-10.8045867817025));
#72917=CARTESIAN_POINT('Ctrl Pts',(-17.192062284342,-20.4025772282142,-10.8050389433295));
#72918=CARTESIAN_POINT('Ctrl Pts',(-17.2001402234296,-20.4111026912632,
-10.8057444727771));
#72919=CARTESIAN_POINT('Ctrl Pts',(-17.2030246197794,-20.4141288801937,
-10.8059962929739));
#72920=CARTESIAN_POINT('Ctrl Pts',(-17.2083844745054,-20.4197189683043,
-10.8064640846992));
#72921=CARTESIAN_POINT('Ctrl Pts',(-17.2108574504169,-20.4222851677875,
-10.8066798649331));
#72922=CARTESIAN_POINT('Ctrl Pts',(-17.216455278627,-20.4280647373772,-10.8071681802184));
#72923=CARTESIAN_POINT('Ctrl Pts',(-17.219583845293,-20.4312744166662,-10.807441003048));
#72924=CARTESIAN_POINT('Ctrl Pts',(-17.2288257878519,-20.4406959231759,
-10.8082465997509));
#72925=CARTESIAN_POINT('Ctrl Pts',(-17.2349672719974,-20.4468798730914,
-10.8087815076653));
#72926=CARTESIAN_POINT('Ctrl Pts',(-17.2789207686384,-20.4905940675539,
-10.8126055245112));
#72927=CARTESIAN_POINT('Ctrl Pts',(-17.3180962975981,-20.5267199583551,
-10.8159914478675));
#72928=CARTESIAN_POINT('Ctrl Pts',(-17.3723156933874,-20.5730585810309,
-10.8206007893428));
#72929=CARTESIAN_POINT('Ctrl Pts',(-17.3861921526224,-20.584614178082,-10.821774126052));
#72930=CARTESIAN_POINT('Ctrl Pts',(-17.4376053551246,-20.6263262087608,
-10.8260938079698));
#72931=CARTESIAN_POINT('Ctrl Pts',(-17.4760193957113,-20.6553766160652,
-10.8292679942957));
#72932=CARTESIAN_POINT('Ctrl Pts',(-17.6048294285987,-20.7460531032254,
-10.8396736914859));
#72933=CARTESIAN_POINT('Ctrl Pts',(-17.6990215663492,-20.8019934660045,
-10.8469061992004));
#72934=CARTESIAN_POINT('Ctrl Pts',(-17.8465280207515,-20.8747891520258,
-10.857479235492));
#72935=CARTESIAN_POINT('Ctrl Pts',(-17.8968715958033,-20.8972355880089,
-10.8609681432704));
#72936=CARTESIAN_POINT('Ctrl Pts',(-17.9798872212718,-20.9304285466725,
-10.8665253906586));
#72937=CARTESIAN_POINT('Ctrl Pts',(-18.0120433432207,-20.9423880022128,
-10.8686321634593));
#72938=CARTESIAN_POINT('Ctrl Pts',(-18.0546963311517,-20.9570816302145,
-10.8713685909166));
#72939=CARTESIAN_POINT('Ctrl Pts',(-18.0649421710351,-20.9605236982969,
-10.8720215847374));
#72940=CARTESIAN_POINT('Ctrl Pts',(-18.0817695475518,-20.9660337680627,
-10.8730870714796));
#72941=CARTESIAN_POINT('Ctrl Pts',(-18.0883355333232,-20.9681483031316,
-10.8735010937725));
#72942=CARTESIAN_POINT('Ctrl Pts',(-18.1010673092143,-20.9721799173819,
-10.8743006074492));
#72943=CARTESIAN_POINT('Ctrl Pts',(-18.10723175743,-20.9741009522746,-10.8746862251603));
#72944=CARTESIAN_POINT('Ctrl Pts',(-18.1214882355998,-20.9784722600781,
-10.8755746517272));
#72945=CARTESIAN_POINT('Ctrl Pts',(-18.1295863827775,-20.980902330048,-10.8760767944877));
#72946=CARTESIAN_POINT('Ctrl Pts',(-18.1514104520049,-20.9873089753633,
-10.8774234279941));
#72947=CARTESIAN_POINT('Ctrl Pts',(-18.165162588493,-20.9911952385216,-10.8782649771697));
#72948=CARTESIAN_POINT('Ctrl Pts',(-18.2917245321447,-21.0255808407728,
-10.8859481709596));
#72949=CARTESIAN_POINT('Ctrl Pts',(-18.40684581723,-21.0468318545523,-10.8924729976926));
#72950=CARTESIAN_POINT('Ctrl Pts',(-18.6851915739438,-21.074693681077,-10.9077869288836));
#72951=CARTESIAN_POINT('Ctrl Pts',(-18.848546917264,-21.0721598589193,-10.9163926288912));
#72952=CARTESIAN_POINT('Ctrl Pts',(-19.0420772806209,-21.0467137523404,
-10.9276020963078));
#72953=CARTESIAN_POINT('Ctrl Pts',(-19.0740756661868,-21.0417573060092,
-10.9294907074751));
#72954=CARTESIAN_POINT('Ctrl Pts',(-19.1130639760767,-21.0347990264385,
-10.9318488356548));
#72955=CARTESIAN_POINT('Ctrl Pts',(-19.1201754921969,-21.0334921975084,
-10.9322812936415));
#72956=CARTESIAN_POINT('Ctrl Pts',(-19.1313162829863,-21.0313858816296,
-10.932962633488));
#72957=CARTESIAN_POINT('Ctrl Pts',(-19.1353502400238,-21.0306110404835,
-10.9332101339289));
#72958=CARTESIAN_POINT('Ctrl Pts',(-19.1428880004036,-21.0291404295187,
-10.9336741375203));
#72959=CARTESIAN_POINT('Ctrl Pts',(-19.1463923064997,-21.0284475302056,
-10.9338904760341));
#72960=CARTESIAN_POINT('Ctrl Pts',(-19.1543899819773,-21.0268451220722,
-10.9343856275422));
#72961=CARTESIAN_POINT('Ctrl Pts',(-19.1588821457535,-21.0259298876386,
-10.9346647634294));
#72962=CARTESIAN_POINT('Ctrl Pts',(-19.1705975386467,-21.0235033306079,
-10.935395332013));
#72963=CARTESIAN_POINT('Ctrl Pts',(-19.1778158289252,-21.021968832088,-10.9358480386525));
#72964=CARTESIAN_POINT('Ctrl Pts',(-19.2250032895863,-21.0116793339687,
-10.9388236899474));
#72965=CARTESIAN_POINT('Ctrl Pts',(-19.2647167027151,-21.0018054699887,
-10.9414041654556));
#72966=CARTESIAN_POINT('Ctrl Pts',(-19.3142212966261,-20.9879622664121,
-10.9446963827874));
#72967=CARTESIAN_POINT('Ctrl Pts',(-19.324305351243,-20.9850614080953,-10.9453709994192));
#72968=CARTESIAN_POINT('Ctrl Pts',(-19.3350136213566,-20.9818945985568,
-10.9460913570241));
#72969=CARTESIAN_POINT('Ctrl Pts',(-19.3356598796412,-20.9817031417266,
-10.9461348470336));
#72970=CARTESIAN_POINT('Ctrl Pts',(-19.3407296351053,-20.9801985705268,
-10.9464761375737));
#72971=CARTESIAN_POINT('Ctrl Pts',(-19.3451488947369,-20.9788713130255,
-10.9467743596194));
#72972=CARTESIAN_POINT('Ctrl Pts',(-19.3733140799957,-20.9703118395231,
-10.9486794861855));
#72973=CARTESIAN_POINT('Ctrl Pts',(-19.3969350472084,-20.9626770591781,
-10.9502975271165));
#72974=CARTESIAN_POINT('Ctrl Pts',(-19.457534237769,-20.9419062439879,-10.9544929616215));
#72975=CARTESIAN_POINT('Ctrl Pts',(-19.4942912559967,-20.9281542829556,
-10.9570808584803));
#72976=CARTESIAN_POINT('Ctrl Pts',(-19.6319039834722,-20.8722610513795,
-10.9668925590682));
#72977=CARTESIAN_POINT('Ctrl Pts',(-19.7298347209471,-20.8233499794817,
-10.9741189015601));
#72978=CARTESIAN_POINT('Ctrl Pts',(-19.8707066194332,-20.7387880145052,
-10.9846789909834));
#72979=CARTESIAN_POINT('Ctrl Pts',(-19.9167399858445,-20.708655996465,-10.9881611598825));
#72980=CARTESIAN_POINT('Ctrl Pts',(-19.9894591996748,-20.6569001770201,
-10.9937089293397));
#72981=CARTESIAN_POINT('Ctrl Pts',(-20.0168825458729,-20.6363618983359,
-10.9958127998496));
#72982=CARTESIAN_POINT('Ctrl Pts',(-20.0522837221869,-20.6084823364114,
-10.9985460660424));
#72983=CARTESIAN_POINT('Ctrl Pts',(-20.0607195893577,-20.6017335666755,
-10.9991987335007));
#72984=CARTESIAN_POINT('Ctrl Pts',(-20.0744558866247,-20.5905708961939,
-11.0002638242202));
#72985=CARTESIAN_POINT('Ctrl Pts',(-20.0797869828508,-20.5861952038791,
-11.0006777746594));
#72986=CARTESIAN_POINT('Ctrl Pts',(-20.0900678101864,-20.5776724116351,
-11.0014772439116));
#72987=CARTESIAN_POINT('Ctrl Pts',(-20.0950201310551,-20.573528568994,-11.0018628885576));
#72988=CARTESIAN_POINT('Ctrl Pts',(-20.1064149699122,-20.5639049852794,
-11.0027515120329));
#72989=CARTESIAN_POINT('Ctrl Pts',(-20.1128437919051,-20.5584091421238,
-11.0032538238192));
#72990=CARTESIAN_POINT('Ctrl Pts',(-20.1300532702657,-20.5435177529472,
-11.0046012100195));
#72991=CARTESIAN_POINT('Ctrl Pts',(-20.1407720671548,-20.5340511551088,
-11.0054433376549));
#72992=CARTESIAN_POINT('Ctrl Pts',(-20.2387839559125,-20.4457054821749,
-11.0131734110647));
#72993=CARTESIAN_POINT('Ctrl Pts',(-20.3194606398749,-20.3597822000834,
-11.0197398870946));
#72994=CARTESIAN_POINT('Ctrl Pts',(-20.4942610015816,-20.1394080997281,
-11.0351344074215));
#72995=CARTESIAN_POINT('Ctrl Pts',(-20.5807193464566,-19.9998893516795,
-11.0437795021006));
#72996=CARTESIAN_POINT('Ctrl Pts',(-20.66341921337,-19.8237747121326,-11.0549700245056));
#72997=CARTESIAN_POINT('Ctrl Pts',(-20.675974861148,-19.7954352730716,-11.0567799147819));
#72998=CARTESIAN_POINT('Ctrl Pts',(-20.690648753905,-19.7602484381654,-11.0590503946498));
#72999=CARTESIAN_POINT('Ctrl Pts',(-20.6933610187251,-19.7536509707836,
-11.05947709945));
#73000=CARTESIAN_POINT('Ctrl Pts',(-20.6975744495108,-19.743252853983,-11.0601513689701));
#73001=CARTESIAN_POINT('Ctrl Pts',(-20.6990980710783,-19.7394612803831,
-11.0603975992514));
#73002=CARTESIAN_POINT('Ctrl Pts',(-20.7019342811529,-19.7323438022282,
-11.0608605435095));
#73003=CARTESIAN_POINT('Ctrl Pts',(-20.7032494244389,-19.7290189754961,
-11.0610771008679));
#73004=CARTESIAN_POINT('Ctrl Pts',(-20.7062437524804,-19.7213925553081,
-11.0615745113123));
#73005=CARTESIAN_POINT('Ctrl Pts',(-20.7079172851563,-19.7170888012446,
-11.0618556986588));
#73006=CARTESIAN_POINT('Ctrl Pts',(-20.7130574312923,-19.70374097718,-11.0627292153072));
#73007=CARTESIAN_POINT('Ctrl Pts',(-20.7164760101577,-19.6946787152548,
-11.0633243042981));
#73008=CARTESIAN_POINT('Ctrl Pts',(-20.7207530624095,-19.6831007664952,
-11.0640868798659));
#73009=CARTESIAN_POINT('Ctrl Pts',(-20.7216691884613,-19.6806063806669,
-11.0642513062267));
#73010=CARTESIAN_POINT('Ctrl Pts',(-20.7225805818558,-19.6781103700305,
-11.0644159698366));
#73011=CARTESIAN_POINT('',(-20.8509993992249,-18.9535948922217,-10.0879364584982));
#73012=CARTESIAN_POINT('Ctrl Pts',(-20.7225805823871,-19.6781103685755,
-10.8441190550425));
#73013=CARTESIAN_POINT('Ctrl Pts',(-20.721654332156,-19.68064706727,-10.8439718791398));
#73014=CARTESIAN_POINT('Ctrl Pts',(-20.7207231989508,-19.6831820734091,
-10.8438247431562));
#73015=CARTESIAN_POINT('Ctrl Pts',(-20.66234998667,-19.8411681008426,-10.834651040078));
#73016=CARTESIAN_POINT('Ctrl Pts',(-20.5868669710953,-19.9893140896377,
-10.8258505888223));
#73017=CARTESIAN_POINT('Ctrl Pts',(-20.4871421897505,-20.1387506012441,
-10.8152892080054));
#73018=CARTESIAN_POINT('Ctrl Pts',(-20.4792655355707,-20.1503040991621,
-10.8144605478709));
#73019=CARTESIAN_POINT('Ctrl Pts',(-20.4681194470797,-20.1663101908851,
-10.8132942461161));
#73020=CARTESIAN_POINT('Ctrl Pts',(-20.464945967379,-20.1708295831989,-10.812962876718));
#73021=CARTESIAN_POINT('Ctrl Pts',(-20.4598136870831,-20.1780780571108,
-10.8124279962897));
#73022=CARTESIAN_POINT('Ctrl Pts',(-20.4578659850139,-20.1808150186255,
-10.8122252432122));
#73023=CARTESIAN_POINT('Ctrl Pts',(-20.4537748168611,-20.1865351648408,
-10.8117998205916));
#73024=CARTESIAN_POINT('Ctrl Pts',(-20.4516300984774,-20.1895174091799,
-10.8115770617094));
#73025=CARTESIAN_POINT('Ctrl Pts',(-20.4464076162739,-20.1967395734038,
-10.8110352940034));
#73026=CARTESIAN_POINT('Ctrl Pts',(-20.4433218642905,-20.2009736637648,
-10.8107157372564));
#73027=CARTESIAN_POINT('Ctrl Pts',(-20.4323912722236,-20.2158556110821,
-10.8095858413374));
#73028=CARTESIAN_POINT('Ctrl Pts',(-20.4244625861269,-20.2264411103798,
-10.8087699648383));
#73029=CARTESIAN_POINT('Ctrl Pts',(-20.3764348919687,-20.2893255912705,
-10.8038532172211));
#73030=CARTESIAN_POINT('Ctrl Pts',(-20.3340141567129,-20.3397986648666,
-10.7996154829477));
#73031=CARTESIAN_POINT('Ctrl Pts',(-20.2240817568495,-20.4588479687894,
-10.7890378447767));
#73032=CARTESIAN_POINT('Ctrl Pts',(-20.1541137448145,-20.5249625621451,
-10.7826421740993));
#73033=CARTESIAN_POINT('Ctrl Pts',(-19.9712621148261,-20.6755654935763,
-10.7670586349167));
#73034=CARTESIAN_POINT('Ctrl Pts',(-19.8539618898259,-20.7539972784858,
-10.7580100967457));
#73035=CARTESIAN_POINT('Ctrl Pts',(-19.7171141005304,-20.8269346200798,
-10.7485414479407));
#73036=CARTESIAN_POINT('Ctrl Pts',(-19.7044367141368,-20.8335275081182,
-10.747673517477));
#73037=CARTESIAN_POINT('Ctrl Pts',(-19.6841535539931,-20.8438162434527,
-10.7462992672034));
#73038=CARTESIAN_POINT('Ctrl Pts',(-19.6765908805431,-20.8475956610821,
-10.7457900197118));
#73039=CARTESIAN_POINT('Ctrl Pts',(-19.6632128770887,-20.8541814103305,
-10.7448946568446));
#73040=CARTESIAN_POINT('Ctrl Pts',(-19.65740700647,-20.8570066116918,-10.7445078854125));
#73041=CARTESIAN_POINT('Ctrl Pts',(-19.6453717578922,-20.8627951494897,
-10.7437098137997));
#73042=CARTESIAN_POINT('Ctrl Pts',(-19.6391406324191,-20.865754692136,-10.7432986490364));
#73043=CARTESIAN_POINT('Ctrl Pts',(-19.6231088296308,-20.8732733601876,
-10.7422459109548));
#73044=CARTESIAN_POINT('Ctrl Pts',(-19.6132874229279,-20.8777880127195,
-10.7416058791007));
#73045=CARTESIAN_POINT('Ctrl Pts',(-19.5721500376953,-20.896317513263,-10.7389449895684));
#73046=CARTESIAN_POINT('Ctrl Pts',(-19.5405292481989,-20.909645740814,-10.7369476656899));
#73047=CARTESIAN_POINT('Ctrl Pts',(-19.457306174465,-20.9423654379907,-10.731802969803));
#73048=CARTESIAN_POINT('Ctrl Pts',(-19.4052450524024,-20.9605211285955,
-10.7286949992077));
#73049=CARTESIAN_POINT('Ctrl Pts',(-19.2479505448434,-21.0085752724312,
-10.7195498706312));
#73050=CARTESIAN_POINT('Ctrl Pts',(-19.1410481739847,-21.0323748894513,
-10.7136614396477));
#73051=CARTESIAN_POINT('Ctrl Pts',(-18.9869104505298,-21.0543493171957,
-10.7051846535349));
#73052=CARTESIAN_POINT('Ctrl Pts',(-18.9408337330223,-21.0593812909741,
-10.7026507573554));
#73053=CARTESIAN_POINT('Ctrl Pts',(-18.8732966600446,-21.0645205820013,
-10.6988935352125));
#73054=CARTESIAN_POINT('Ctrl Pts',(-18.8519399092396,-21.0658204521351,
-10.6976990983847));
#73055=CARTESIAN_POINT('Ctrl Pts',(-18.7787684009524,-21.0691616723124,
-10.6935745735534));
#73056=CARTESIAN_POINT('Ctrl Pts',(-18.7269041839199,-21.0696228328302,
-10.6905959948421));
#73057=CARTESIAN_POINT('Ctrl Pts',(-18.6664282755531,-21.0679390291251,
-10.687005316025));
#73058=CARTESIAN_POINT('Ctrl Pts',(-18.657778129181,-21.0676450868561,-10.6864889123011));
#73059=CARTESIAN_POINT('Ctrl Pts',(-18.6446645796776,-21.067118946185,-10.6857014564131));
#73060=CARTESIAN_POINT('Ctrl Pts',(-18.6401995885298,-21.066925638362,-10.6854325303205));
#73061=CARTESIAN_POINT('Ctrl Pts',(-18.6321760418079,-21.066552807839,-10.6849477675161));
#73062=CARTESIAN_POINT('Ctrl Pts',(-18.6286173011567,-21.0663784387093,
-10.6847322221513));
#73063=CARTESIAN_POINT('Ctrl Pts',(-18.6208737703034,-21.065979427197,-10.6842620372403));
#73064=CARTESIAN_POINT('Ctrl Pts',(-18.6166892555886,-21.065751345594,-10.6840072124888));
#73065=CARTESIAN_POINT('Ctrl Pts',(-18.6049071857032,-21.0650740569778,
-10.6832876809919));
#73066=CARTESIAN_POINT('Ctrl Pts',(-18.5973114260672,-21.064596306608,-10.6828214205683));
#73067=CARTESIAN_POINT('Ctrl Pts',(-18.5512917547967,-21.0614525844054,
-10.6799827382927));
#73068=CARTESIAN_POINT('Ctrl Pts',(-18.5129464670905,-21.0577795262608,
-10.6775592052215));
#73069=CARTESIAN_POINT('Ctrl Pts',(-18.3856271384966,-21.0420681277534,
-10.6693639794191));
#73070=CARTESIAN_POINT('Ctrl Pts',(-18.2973236371973,-21.0254175170392,
-10.6634411578528));
#73071=CARTESIAN_POINT('Ctrl Pts',(-18.0441419775274,-20.9607832913705,
-10.6461741899727));
#73072=CARTESIAN_POINT('Ctrl Pts',(-17.8836741157218,-20.8982996341513,
-10.6349280904655));
#73073=CARTESIAN_POINT('Ctrl Pts',(-17.7119984076849,-20.806115065783,-10.6229309439354));
#73074=CARTESIAN_POINT('Ctrl Pts',(-17.6916898153342,-20.7947749397357,
-10.6215108837775));
#73075=CARTESIAN_POINT('Ctrl Pts',(-17.663276567896,-20.7782892165825,-10.619522198383));
#73076=CARTESIAN_POINT('Ctrl Pts',(-17.6550142637645,-20.7734199835285,
-10.6189436709301));
#73077=CARTESIAN_POINT('Ctrl Pts',(-17.6416585403609,-20.7654262691874,
-10.6180080323445));
#73078=CARTESIAN_POINT('Ctrl Pts',(-17.6365448286014,-20.7623361141328,
-10.6176496770886));
#73079=CARTESIAN_POINT('Ctrl Pts',(-17.6258802748347,-20.7558298574641,
-10.6169020669863));
#73080=CARTESIAN_POINT('Ctrl Pts',(-17.6203319814758,-20.7524096828114,
-10.6165129665454));
#73081=CARTESIAN_POINT('Ctrl Pts',(-17.6071924962542,-20.7442260359152,
-10.6155910864694));
#73082=CARTESIAN_POINT('Ctrl Pts',(-17.5996155436419,-20.739439851644,-10.6150591515117));
#73083=CARTESIAN_POINT('Ctrl Pts',(-17.5742945447087,-20.7232193091537,
-10.6132802021167));
#73084=CARTESIAN_POINT('Ctrl Pts',(-17.5566908130909,-20.7115674781159,
-10.6120412841322));
#73085=CARTESIAN_POINT('Ctrl Pts',(-17.462462336009,-20.6471507386989,-10.6053928432974));
#73086=CARTESIAN_POINT('Ctrl Pts',(-17.3892005001075,-20.5896389295884,
-10.6001689098512));
#73087=CARTESIAN_POINT('Ctrl Pts',(-17.2048003946038,-20.4241343864209,
-10.5865236892977));
#73088=CARTESIAN_POINT('Ctrl Pts',(-17.1013352948134,-20.3084772792071,
-10.578341240394));
#73089=CARTESIAN_POINT('Ctrl Pts',(-16.9802264995808,-20.138947380487,-10.5666271778609));
#73090=CARTESIAN_POINT('Ctrl Pts',(-16.9507222853145,-20.094140592561,-10.5635502962915));
#73091=CARTESIAN_POINT('Ctrl Pts',(-16.9184272112633,-20.0407887090463,
-10.5598495256133));
#73092=CARTESIAN_POINT('Ctrl Pts',(-16.9139472470223,-20.0332832073824,
-10.5593280725652));
#73093=CARTESIAN_POINT('Ctrl Pts',(-16.9072378062841,-20.0218827164531,
-10.5585344210374));
#73094=CARTESIAN_POINT('Ctrl Pts',(-16.904973961376,-20.0180079214236,-10.5582643991173));
#73095=CARTESIAN_POINT('Ctrl Pts',(-16.9009342368253,-20.011042780965,-10.5577784729938));
#73096=CARTESIAN_POINT('Ctrl Pts',(-16.8991538272415,-20.0079551250207,
-10.5575628663861));
#73097=CARTESIAN_POINT('Ctrl Pts',(-16.8953040930042,-20.0012396315514,
-10.5570934983962));
#73098=CARTESIAN_POINT('Ctrl Pts',(-16.8932377311395,-19.9976102101956,
-10.5568395570042));
#73099=CARTESIAN_POINT('Ctrl Pts',(-16.8874685550356,-19.9874069486464,
-10.5561249586191));
#73100=CARTESIAN_POINT('Ctrl Pts',(-16.8837901684364,-19.9808194699733,
-10.5556627811539));
#73101=CARTESIAN_POINT('Ctrl Pts',(-16.8621082588388,-19.9414978349402,
-10.5528997849538));
#73102=CARTESIAN_POINT('Ctrl Pts',(-16.8449397535161,-19.9083135704699,
-10.5505509047069));
#73103=CARTESIAN_POINT('Ctrl Pts',(-16.7915325222157,-19.7980290572225,
-10.5427306927185));
#73104=CARTESIAN_POINT('Ctrl Pts',(-16.7590691122222,-19.7191969686125,
-10.5371218810942));
#73105=CARTESIAN_POINT('Ctrl Pts',(-16.6736890748013,-19.4701861005766,
-10.5197317279115));
#73106=CARTESIAN_POINT('Ctrl Pts',(-16.6374050927338,-19.2950921422355,
-10.5080297421229));
#73107=CARTESIAN_POINT('Ctrl Pts',(-16.6216974500578,-19.0947803478442,
-10.4956647963491));
#73108=CARTESIAN_POINT('Ctrl Pts',(-16.6202828609828,-19.0720342040855,
-10.4942738524237));
#73109=CARTESIAN_POINT('Ctrl Pts',(-16.6187986907307,-19.0397662431442,
-10.4923185681888));
#73110=CARTESIAN_POINT('Ctrl Pts',(-16.6184256628598,-19.0302605956026,
-10.4917447694746));
#73111=CARTESIAN_POINT('Ctrl Pts',(-16.6179231307851,-19.0147950176111,
-10.4908146978918));
#73112=CARTESIAN_POINT('Ctrl Pts',(-16.6177547077915,-19.0088365639154,
-10.4904572099336));
#73113=CARTESIAN_POINT('Ctrl Pts',(-16.6174545212065,-18.9963494661293,
-10.4897097598633));
#73114=CARTESIAN_POINT('Ctrl Pts',(-16.6173277932303,-18.9898207550052,
-10.4893199594034));
#73115=CARTESIAN_POINT('Ctrl Pts',(-16.6170978152185,-18.9742634891722,
-10.4883934221738));
#73116=CARTESIAN_POINT('Ctrl Pts',(-16.6170221135093,-18.9652346075889,
-10.4878575533742));
#73117=CARTESIAN_POINT('Ctrl Pts',(-16.6169614563799,-18.9346999186841,
-10.4860513879421));
#73118=CARTESIAN_POINT('Ctrl Pts',(-16.6172464316565,-18.9131944715482,
-10.4847895354095));
#73119=CARTESIAN_POINT('Ctrl Pts',(-16.6229818787195,-18.7119289702551,
-10.4730664950018));
#73120=CARTESIAN_POINT('Ctrl Pts',(-16.650988260201,-18.5335497020633,-10.4634059639935));
#73121=CARTESIAN_POINT('Ctrl Pts',(-16.7347415328079,-18.2455500022279,
-10.4470815795015));
#73122=CARTESIAN_POINT('Ctrl Pts',(-16.7780138208059,-18.1333329819364,
-10.440492433379));
#73123=CARTESIAN_POINT('Ctrl Pts',(-16.8347150170204,-18.016855095654,-10.432814929758));
#73124=CARTESIAN_POINT('Ctrl Pts',(-16.8389349183148,-18.0083328090676,
-10.4322480843172));
#73125=CARTESIAN_POINT('Ctrl Pts',(-16.8452734803941,-17.9957457755526,
-10.4314028597307));
#73126=CARTESIAN_POINT('Ctrl Pts',(-16.8473482214746,-17.9916588765876,
-10.4311271614003));
#73127=CARTESIAN_POINT('Ctrl Pts',(-16.8510635049801,-17.9843988860813,
-10.4306351043593));
#73128=CARTESIAN_POINT('Ctrl Pts',(-16.8526988225738,-17.9812231772852,
-10.4304190754897));
#73129=CARTESIAN_POINT('Ctrl Pts',(-16.8562323263675,-17.9744037422464,
-10.4299534632163));
#73130=CARTESIAN_POINT('Ctrl Pts',(-16.8581330563605,-17.970761451832,-10.4297037248402));
#73131=CARTESIAN_POINT('Ctrl Pts',(-16.8634097332128,-17.9607213392477,
-10.4290124493867));
#73132=CARTESIAN_POINT('Ctrl Pts',(-16.8668078519805,-17.9543353226877,
-10.4285695444434));
#73133=CARTESIAN_POINT('Ctrl Pts',(-16.8856168563481,-17.9194206384387,
-10.4261308510631));
#73134=CARTESIAN_POINT('Ctrl Pts',(-16.9016480041505,-17.8912331639775,
-10.4240989740089));
#73135=CARTESIAN_POINT('Ctrl Pts',(-17.0020305028812,-17.7238006088581,
-10.41169536643));
#73136=CARTESIAN_POINT('Ctrl Pts',(-17.1015653443001,-17.5943000723529,
-10.4007319227682));
#73137=CARTESIAN_POINT('Ctrl Pts',(-17.2963461628739,-17.3936369333862,
-10.3824650355408));
#73138=CARTESIAN_POINT('Ctrl Pts',(-17.3845492722723,-17.3166607229697,
-10.3750213987216));
#73139=CARTESIAN_POINT('Ctrl Pts',(-17.4901699542042,-17.2388801006792,
-10.3670122466832));
#73140=CARTESIAN_POINT('Ctrl Pts',(-17.5017556359537,-17.2305277187122,
-10.3661447298444));
#73141=CARTESIAN_POINT('Ctrl Pts',(-17.5203312227918,-17.2174197794686,
-10.3647710086347));
#73142=CARTESIAN_POINT('Ctrl Pts',(-17.5272664644299,-17.2125878522914,
-10.3642618800883));
#73143=CARTESIAN_POINT('Ctrl Pts',(-17.5395499552708,-17.2041385137033,
-10.3633666555635));
#73144=CARTESIAN_POINT('Ctrl Pts',(-17.5448861281116,-17.2005038150918,
-10.3629799041664));
#73145=CARTESIAN_POINT('Ctrl Pts',(-17.555958479747,-17.1930358810124,-10.3621818060875));
#73146=CARTESIAN_POINT('Ctrl Pts',(-17.5616969421382,-17.1892061556762,
-10.3617705951576));
#73147=CARTESIAN_POINT('Ctrl Pts',(-17.5764770268571,-17.1794463392741,
-10.3607175984647));
#73148=CARTESIAN_POINT('Ctrl Pts',(-17.5855456163395,-17.1735572967557,
-10.3600773556533));
#73149=CARTESIAN_POINT('Ctrl Pts',(-17.6236016868468,-17.1492565847232,
-10.357414414779));
#73150=CARTESIAN_POINT('Ctrl Pts',(-17.6529908205066,-17.131481506216,-10.3554152968543));
#73151=CARTESIAN_POINT('Ctrl Pts',(-17.7306991380011,-17.0870277633216,
-10.3502649343218));
#73152=CARTESIAN_POINT('Ctrl Pts',(-17.7796527953812,-17.061509025676,-10.3471532050509));
#73153=CARTESIAN_POINT('Ctrl Pts',(-18.0001640608131,-16.9573114816709,
-10.3335928911971));
#73154=CARTESIAN_POINT('Ctrl Pts',(-18.1807674339952,-16.8998749470545,
-10.3237454457231));
#73155=CARTESIAN_POINT('Ctrl Pts',(-18.4072158569911,-16.8599663968284,
-10.3106716474144));
#73156=CARTESIAN_POINT('Ctrl Pts',(-18.4480604320674,-16.8539936769848,
-10.3082823569198));
#73157=CARTESIAN_POINT('Ctrl Pts',(-18.4963994698329,-16.8483627376973,
-10.3053907873153));
#73158=CARTESIAN_POINT('Ctrl Pts',(-18.5037529616296,-16.8475451915094,
-10.3049491761383));
#73159=CARTESIAN_POINT('Ctrl Pts',(-18.5156752363866,-16.8462829325157,
-10.304230158663));
#73160=CARTESIAN_POINT('Ctrl Pts',(-18.5202415175733,-16.8458144951164,
-10.3039540526395));
#73161=CARTESIAN_POINT('Ctrl Pts',(-18.5283645190566,-16.8450078752761,
-10.3034615490718));
#73162=CARTESIAN_POINT('Ctrl Pts',(-18.5319206080349,-16.8446638417687,
-10.3032454836792));
#73163=CARTESIAN_POINT('Ctrl Pts',(-18.5395634333902,-16.8439439609681,
-10.3027801130099));
#73164=CARTESIAN_POINT('Ctrl Pts',(-18.5436503363709,-16.8435710002399,
-10.3025306544487));
#73165=CARTESIAN_POINT('Ctrl Pts',(-18.5549236141006,-16.8425752726991,
-10.3018409237011));
#73166=CARTESIAN_POINT('Ctrl Pts',(-18.562112048801,-16.8419773553544,-10.3013992935025));
#73167=CARTESIAN_POINT('Ctrl Pts',(-18.6013323208737,-16.8389168513302,
-10.2989803359217));
#73168=CARTESIAN_POINT('Ctrl Pts',(-18.633412144967,-16.8371470665829,-10.2969675913487));
#73169=CARTESIAN_POINT('Ctrl Pts',(-18.8284837672567,-16.8308334396913,
-10.2845703249421));
#73170=CARTESIAN_POINT('Ctrl Pts',(-18.9915088627262,-16.8444033070309,
-10.2735892285581));
#73171=CARTESIAN_POINT('Ctrl Pts',(-19.2659681080618,-16.8995952760549,
-10.2553020994591));
#73172=CARTESIAN_POINT('Ctrl Pts',(-19.3784846450023,-16.9320983726147,
-10.2478551001261));
#73173=CARTESIAN_POINT('Ctrl Pts',(-19.5011217458905,-16.9788254618589,
-10.2398416205954));
#73174=CARTESIAN_POINT('Ctrl Pts',(-19.5144342696115,-16.9840528722652,
-10.2389729004162));
#73175=CARTESIAN_POINT('Ctrl Pts',(-19.5355341451213,-16.9925859160875,
-10.237597640089));
#73176=CARTESIAN_POINT('Ctrl Pts',(-19.543356242556,-16.9958039428756,-10.2370881655599));
#73177=CARTESIAN_POINT('Ctrl Pts',(-19.5571157825931,-17.0015613044551,
-10.2361925385826));
#73178=CARTESIAN_POINT('Ctrl Pts',(-19.5630612466798,-17.0040810727035,
-10.2358057288595));
#73179=CARTESIAN_POINT('Ctrl Pts',(-19.5744704106973,-17.0089781292245,
-10.2350637801813));
#73180=CARTESIAN_POINT('Ctrl Pts',(-19.5799357776103,-17.0113513551275,
-10.2347085074487));
#73181=CARTESIAN_POINT('Ctrl Pts',(-19.594340085058,-17.0176785493396,-10.2337725061402));
#73182=CARTESIAN_POINT('Ctrl Pts',(-19.6032618547738,-17.0216714349256,
-10.2331931130482));
#73183=CARTESIAN_POINT('Ctrl Pts',(-19.6363015689364,-17.0367336824467,
-10.231048471716));
#73184=CARTESIAN_POINT('Ctrl Pts',(-19.6602390128667,-17.0481947125768,
-10.2294967117845));
#73185=CARTESIAN_POINT('Ctrl Pts',(-19.7190604166622,-17.0777299985423,
-10.2256838278797));
#73186=CARTESIAN_POINT('Ctrl Pts',(-19.7536693107868,-17.0963311657396,
-10.2234407683219));
#73187=CARTESIAN_POINT('Ctrl Pts',(-19.8816272910708,-17.1697659698881,
-10.2151169071897));
#73188=CARTESIAN_POINT('Ctrl Pts',(-19.9712461359685,-17.2307705860135,
-10.209233383477));
#73189=CARTESIAN_POINT('Ctrl Pts',(-20.1621976467807,-17.3834047618063,
-10.1959581259965));
#73190=CARTESIAN_POINT('Ctrl Pts',(-20.260117338126,-17.4785024137405,-10.1886009569423));
#73191=CARTESIAN_POINT('Ctrl Pts',(-20.3583115020396,-17.5942280116429,
-10.1797012825132));
#73192=CARTESIAN_POINT('Ctrl Pts',(-20.3682778060191,-17.6062404937221,
-10.1787778879968));
#73193=CARTESIAN_POINT('Ctrl Pts',(-20.3817499242634,-17.6228489283591,
-10.1775000223475));
#73194=CARTESIAN_POINT('Ctrl Pts',(-20.3853713727367,-17.6273510005747,
-10.1771535122544));
#73195=CARTESIAN_POINT('Ctrl Pts',(-20.3910999010786,-17.6345325290855,
-10.1766004852127));
#73196=CARTESIAN_POINT('Ctrl Pts',(-20.3932190483917,-17.6372023851,-10.1763948251634));
#73197=CARTESIAN_POINT('Ctrl Pts',(-20.3975850695391,-17.6427303815051,
-10.1759688447163));
#73198=CARTESIAN_POINT('Ctrl Pts',(-20.3998310254622,-17.6455891873776,
-10.1757484594032));
#73199=CARTESIAN_POINT('Ctrl Pts',(-20.4051694785284,-17.6524204839468,
-10.1752216467053));
#73200=CARTESIAN_POINT('Ctrl Pts',(-20.4082551813425,-17.6563982359319,
-10.174914742553));
#73201=CARTESIAN_POINT('Ctrl Pts',(-20.4186340286359,-17.669876511333,-10.1738744286385));
#73202=CARTESIAN_POINT('Ctrl Pts',(-20.4258605716586,-17.6794277067749,
-10.1731365647873));
#73203=CARTESIAN_POINT('Ctrl Pts',(-20.5082076495465,-17.7902056223147,
-10.1645759869468));
#73204=CARTESIAN_POINT('Ctrl Pts',(-20.5742159455847,-17.8978759174788,
-10.1562456568966));
#73205=CARTESIAN_POINT('Ctrl Pts',(-20.6639570531766,-18.0786715880011,
-10.1429069302171));
#73206=CARTESIAN_POINT('Ctrl Pts',(-20.6939937560356,-18.1483444894198,
-10.1379032853588));
#73207=CARTESIAN_POINT('Ctrl Pts',(-20.7344247282807,-18.257973289476,-10.1303131310646));
#73208=CARTESIAN_POINT('Ctrl Pts',(-20.7474992285013,-18.2968715254224,
-10.1276720761972));
#73209=CARTESIAN_POINT('Ctrl Pts',(-20.7623062613021,-18.3455677444204,
-10.1244341970915));
#73210=CARTESIAN_POINT('Ctrl Pts',(-20.7651109235248,-18.3550286512658,
-10.1238082752894));
#73211=CARTESIAN_POINT('Ctrl Pts',(-20.7833788644753,-18.4182708730031,
-10.1196453528436));
#73212=CARTESIAN_POINT('Ctrl Pts',(-20.7967716114792,-18.4726309223956,
-10.1161695253994));
#73213=CARTESIAN_POINT('Ctrl Pts',(-20.8104073081852,-18.5392454074478,
-10.112030449285));
#73214=CARTESIAN_POINT('Ctrl Pts',(-20.8127188682339,-18.5510492057949,
-10.1113015163257));
#73215=CARTESIAN_POINT('Ctrl Pts',(-20.8163752168606,-18.5706021797478,
-10.1101013105191));
#73216=CARTESIAN_POINT('Ctrl Pts',(-20.8177776223906,-18.5783401759405,
-10.1096282104574));
#73217=CARTESIAN_POINT('Ctrl Pts',(-20.8202374512184,-18.5923573446946,
-10.1087745383789));
#73218=CARTESIAN_POINT('Ctrl Pts',(-20.8213097188383,-18.5986337857175,
-10.1083934983669));
#73219=CARTESIAN_POINT('Ctrl Pts',(-20.8233364623021,-18.6108283703562,
-10.1076554767596));
#73220=CARTESIAN_POINT('Ctrl Pts',(-20.8242941494265,-18.6167459119008,
-10.1072983966081));
#73221=CARTESIAN_POINT('Ctrl Pts',(-20.8263396785846,-18.6297348062099,
-10.1065168817455));
#73222=CARTESIAN_POINT('Ctrl Pts',(-20.8274168374647,-18.6368077852555,
-10.106092788067));
#73223=CARTESIAN_POINT('Ctrl Pts',(-20.8299772084217,-18.6542123578294,
-10.1050527574227));
#73224=CARTESIAN_POINT('Ctrl Pts',(-20.8314199196078,-18.6645497874455,
-10.104438096375));
#73225=CARTESIAN_POINT('Ctrl Pts',(-20.8449846070162,-18.7672893463057,
-10.0983585509772));
#73226=CARTESIAN_POINT('Ctrl Pts',(-20.851069617783,-18.8603894435261,-10.093091189706));
#73227=CARTESIAN_POINT('Ctrl Pts',(-20.8509993992249,-18.9535948922217,
-10.0879364584982));
#73228=CARTESIAN_POINT('Ctrl Pts',(-20.8509994011068,-18.9535923923061,
-10.0879365967561));
#73229=CARTESIAN_POINT('Ctrl Pts',(-20.850883505645,-19.1076691373228,-10.0794153726715));
#73230=CARTESIAN_POINT('Ctrl Pts',(-20.8339479021024,-19.2612691803274,
-10.0712643188475));
#73231=CARTESIAN_POINT('Ctrl Pts',(-20.7877757711039,-19.4688406968946,
-10.0593982033839));
#73232=CARTESIAN_POINT('Ctrl Pts',(-20.7726928098578,-19.5254541017574,
-10.0560661702904));
#73233=CARTESIAN_POINT('Ctrl Pts',(-20.7515883197402,-19.5932339086432,
-10.0518806465533));
#73234=CARTESIAN_POINT('Ctrl Pts',(-20.7477880301854,-19.6050706748842,
-10.0511423048045));
#73235=CARTESIAN_POINT('Ctrl Pts',(-20.7422787371043,-19.621725042868,-10.0500920839653));
#73236=CARTESIAN_POINT('Ctrl Pts',(-20.7406561150653,-19.6265712368428,
-10.0497851180081));
#73237=CARTESIAN_POINT('Ctrl Pts',(-20.7378448456755,-19.6348675940094,
-10.0492571927926));
#73238=CARTESIAN_POINT('Ctrl Pts',(-20.7366647828737,-19.6383206857942,
-10.0490367396442));
#73239=CARTESIAN_POINT('Ctrl Pts',(-20.7343716263545,-19.644974632166,-10.048610516056));
#73240=CARTESIAN_POINT('Ctrl Pts',(-20.7332597708327,-19.6481758777097,
-10.0484048244984));
#73241=CARTESIAN_POINT('Ctrl Pts',(-20.7302650144133,-19.6567320147411,
-10.0478533928633));
#73242=CARTESIAN_POINT('Ctrl Pts',(-20.7283682704733,-19.6620819814589,
-10.047506842636));
#73243=CARTESIAN_POINT('Ctrl Pts',(-20.7251697799558,-19.6709897494137,
-10.0469269837388));
#73244=CARTESIAN_POINT('Ctrl Pts',(-20.7238799494575,-19.6745518239872,
-10.0466943454164));
#73245=CARTESIAN_POINT('Ctrl Pts',(-20.722580582123,-19.6781103692989,-10.0464611886058));
#73246=CARTESIAN_POINT('Origin',(-18.734,-18.952,0.));
#73247=CARTESIAN_POINT('',(-20.7225807271506,-19.6781099721152,-9.24346982890923));
#73248=CARTESIAN_POINT('',(-20.7225805821191,-19.6781103693095,-9.46634969989166));
#73249=CARTESIAN_POINT('',(-20.7225805821191,-19.6781103693095,0.));
#73250=CARTESIAN_POINT('',(-20.8516083971888,-18.9501065433296,-9.51094371951038));
#73251=CARTESIAN_POINT('Ctrl Pts',(-20.7225805821191,-19.6781103693095,
-9.46634969989166));
#73252=CARTESIAN_POINT('Ctrl Pts',(-20.7472616655809,-19.610516894003,-9.47066128466945));
#73253=CARTESIAN_POINT('Ctrl Pts',(-20.7684942812802,-19.5416581924624,
-9.47497286944723));
#73254=CARTESIAN_POINT('Ctrl Pts',(-20.7861613956308,-19.4719255776385,
-9.47928445422502));
#73255=CARTESIAN_POINT('Ctrl Pts',(-20.8038310616679,-19.4021828912336,
-9.48359666173114));
#73256=CARTESIAN_POINT('Ctrl Pts',(-20.8179340943008,-19.3315665265442,
-9.48790886923727));
#73257=CARTESIAN_POINT('Ctrl Pts',(-20.8284043739734,-19.2604790402619,
-9.4922210767434));
#73258=CARTESIAN_POINT('Ctrl Pts',(-20.8388856820424,-19.1893166771852,
-9.49653782631863));
#73259=CARTESIAN_POINT('Ctrl Pts',(-20.8457265470577,-19.1176826969835,
-9.50085457589386));
#73260=CARTESIAN_POINT('Ctrl Pts',(-20.8489127383039,-19.045984622997,-9.50517132546909));
#73261=CARTESIAN_POINT('Ctrl Pts',(-20.8503329332884,-19.014026326333,-9.50709544917115));
#73262=CARTESIAN_POINT('Ctrl Pts',(-20.8510277144304,-18.9820552992082,
-9.50901957287322));
#73263=CARTESIAN_POINT('Ctrl Pts',(-20.8509991540683,-18.9501074689014,
-9.51094369657528));
#73264=CARTESIAN_POINT('Ctrl Pts',(-20.8516473698352,-18.9501064841217,
-9.51094372097751));
#73265=CARTESIAN_POINT('Ctrl Pts',(-20.8529700774227,-18.8071177722941,
-9.51955279572482));
#73266=CARTESIAN_POINT('Ctrl Pts',(-20.7745204018912,-17.9614816365997,
-9.57055380603263));
#73267=CARTESIAN_POINT('Ctrl Pts',(-19.6371491233128,-16.6173369466333,
-9.66394675190085));
#73268=CARTESIAN_POINT('Ctrl Pts',(-17.2597753314279,-16.928885683341,-9.79112255858232));
#73269=CARTESIAN_POINT('Ctrl Pts',(-16.2349111722559,-19.0965162369476,
-9.91829836526373));
#73270=CARTESIAN_POINT('Ctrl Pts',(-17.5028059015931,-21.1315621128438,
-10.0454741719452));
#73271=CARTESIAN_POINT('Ctrl Pts',(-19.6892757596572,-21.1638770149718,
-10.1614588037971));
#73272=CARTESIAN_POINT('Ctrl Pts',(-20.5391740279707,-20.1636738456026,
-10.2350515000887));
#73273=CARTESIAN_POINT('Ctrl Pts',(-20.7219729237027,-19.6778789621698,
-10.2662522608197));
#73274=CARTESIAN_POINT('Ctrl Pts',(-20.722580582123,-19.6781103692989,-10.0464611886058));
#73275=CARTESIAN_POINT('Ctrl Pts',(-20.7187550915236,-19.6885871461701,
-10.0457747474716));
#73276=CARTESIAN_POINT('Ctrl Pts',(-20.7148469372165,-19.6990333320199,
-10.0450838126525));
#73277=CARTESIAN_POINT('Ctrl Pts',(-20.6549184747011,-19.8554400803251,
-10.0346460290459));
#73278=CARTESIAN_POINT('Ctrl Pts',(-20.5829848665573,-19.9947754284463,
-10.0241696945664));
#73279=CARTESIAN_POINT('Ctrl Pts',(-20.459226806328,-20.1807298986069,-10.0094649923507));
#73280=CARTESIAN_POINT('Ctrl Pts',(-20.4194453519409,-20.2347547271001,
-10.005087012774));
#73281=CARTESIAN_POINT('Ctrl Pts',(-20.3438774955942,-20.3277799833174,
-9.99739792145197));
#73282=CARTESIAN_POINT('Ctrl Pts',(-20.3090674751063,-20.3674996609403,
-9.99406021181886));
#73283=CARTESIAN_POINT('Ctrl Pts',(-20.2576202360407,-20.4219521561615,
-9.98940797716126));
#73284=CARTESIAN_POINT('Ctrl Pts',(-20.2421828076885,-20.4377868761848,
-9.98804521972032));
#73285=CARTESIAN_POINT('Ctrl Pts',(-20.2145560326903,-20.4652502938927,
-9.98566350175101));
#73286=CARTESIAN_POINT('Ctrl Pts',(-20.2024709059035,-20.4769806038585,
-9.98464012615214));
#73287=CARTESIAN_POINT('Ctrl Pts',(-20.1843140782033,-20.4941883431244,
-9.98312940303068));
#73288=CARTESIAN_POINT('Ctrl Pts',(-20.178348770264,-20.4997766130378,-9.98263726626117));
#73289=CARTESIAN_POINT('Ctrl Pts',(-20.1676419638449,-20.5096908908263,
-9.98176135675834));
#73290=CARTESIAN_POINT('Ctrl Pts',(-20.1629129020684,-20.5140301250517,
-9.9813770202822));
#73291=CARTESIAN_POINT('Ctrl Pts',(-20.1536163277823,-20.5224828119447,
-9.98062639583515));
#73292=CARTESIAN_POINT('Ctrl Pts',(-20.1490504928204,-20.5265980073383,
-9.98026003600057));
#73293=CARTESIAN_POINT('Ctrl Pts',(-20.1366409690211,-20.5376851646344,
-9.97927044418196));
#73294=CARTESIAN_POINT('Ctrl Pts',(-20.1287631901906,-20.5446188428548,
-9.9786488209032));
#73295=CARTESIAN_POINT('Ctrl Pts',(-20.0989372486999,-20.5704792951196,
-9.97631954289845));
#73296=CARTESIAN_POINT('Ctrl Pts',(-20.0766521460087,-20.5890138229301,
-9.97462805555531));
#73297=CARTESIAN_POINT('Ctrl Pts',(-20.0515903372689,-20.6090015525466,
-9.97277604555553));
#73298=CARTESIAN_POINT('Ctrl Pts',(-20.0491838352121,-20.6109122706577,
-9.97259871195944));
#73299=CARTESIAN_POINT('Ctrl Pts',(-19.9172692520436,-20.7151825471311,
-9.96290520055451));
#73300=CARTESIAN_POINT('Ctrl Pts',(-19.7762389490106,-20.8020491981962,
-9.95403301223472));
#73301=CARTESIAN_POINT('Ctrl Pts',(-19.548204367267,-20.9080733234487,-9.94034793969889));
#73302=CARTESIAN_POINT('Ctrl Pts',(-19.4677210862196,-20.9396625988341,
-9.93561679888838));
#73303=CARTESIAN_POINT('Ctrl Pts',(-19.3497026771053,-20.9778375961337,
-9.92853371290306));
#73304=CARTESIAN_POINT('Ctrl Pts',(-19.3135640507415,-20.9884706894498,
-9.92634552173695));
#73305=CARTESIAN_POINT('Ctrl Pts',(-19.2698540958267,-21.000073871433,-9.92365477310876));
#73306=CARTESIAN_POINT('Ctrl Pts',(-19.2625343092727,-21.0019750424996,
-9.92320270139751));
#73307=CARTESIAN_POINT('Ctrl Pts',(-19.2511529735457,-21.0048661127848,
-9.92249728223481));
#73308=CARTESIAN_POINT('Ctrl Pts',(-19.2470983289707,-21.0058832924928,
-9.92224548162995));
#73309=CARTESIAN_POINT('Ctrl Pts',(-19.2395813512201,-21.0077454120221,
-9.92177770766564));
#73310=CARTESIAN_POINT('Ctrl Pts',(-19.2361198871982,-21.0085936205404,
-9.92156192548175));
#73311=CARTESIAN_POINT('Ctrl Pts',(-19.2282997756501,-21.0104889666802,
-9.92107358183766));
#73312=CARTESIAN_POINT('Ctrl Pts',(-19.223939959272,-21.0115309974859,-9.92080073245111));
#73313=CARTESIAN_POINT('Ctrl Pts',(-19.2110917941654,-21.014558705917,-9.9199949862861));
#73314=CARTESIAN_POINT('Ctrl Pts',(-19.2025945720958,-21.0165057801839,
-9.91945995430702));
#73315=CARTESIAN_POINT('Ctrl Pts',(-19.1420507203019,-21.0299859190133,
-9.91563371873206));
#73316=CARTESIAN_POINT('Ctrl Pts',(-19.0896011856568,-21.0396009274838,
-9.91224557989896));
#73317=CARTESIAN_POINT('Ctrl Pts',(-19.0096867213254,-21.0511519920042,
-9.90702723502794));
#73318=CARTESIAN_POINT('Ctrl Pts',(-18.9824504918898,-21.0545495291893,
-9.90523891355756));
#73319=CARTESIAN_POINT('Ctrl Pts',(-18.8184280549174,-21.0717787395807,
-9.89443653042584));
#73320=CARTESIAN_POINT('Ctrl Pts',(-18.6806127534488,-21.072788622229,-9.88525203852045));
#73321=CARTESIAN_POINT('Ctrl Pts',(-18.4818913021121,-21.0548500095181,
-9.87235864899197));
#73322=CARTESIAN_POINT('Ctrl Pts',(-18.4203814790917,-21.0465599832269,
-9.86841236794707));
#73323=CARTESIAN_POINT('Ctrl Pts',(-18.3225554016999,-21.0289683844883,
-9.86221849707654));
#73324=CARTESIAN_POINT('Ctrl Pts',(-18.2859707463055,-21.0213850280445,
-9.85992058481192));
#73325=CARTESIAN_POINT('Ctrl Pts',(-18.2387546380831,-21.0102869682285,
-9.85697705777438));
#73326=CARTESIAN_POINT('Ctrl Pts',(-18.227925411775,-21.0076511695017,-9.85630345965948));
#73327=CARTESIAN_POINT('Ctrl Pts',(-18.2103561707791,-21.003227620575,-9.85521295884289));
#73328=CARTESIAN_POINT('Ctrl Pts',(-18.2036033899213,-21.0014919002323,
-9.85479438597461));
#73329=CARTESIAN_POINT('Ctrl Pts',(-18.1906396387028,-20.9980913623198,
-9.85399186669419));
#73330=CARTESIAN_POINT('Ctrl Pts',(-18.1844274467638,-20.9964315482125,
-9.85360776346931));
#73331=CARTESIAN_POINT('Ctrl Pts',(-18.1702292296614,-20.9925685841567,
-9.85273089308057));
#73332=CARTESIAN_POINT('Ctrl Pts',(-18.1622483489522,-20.990346800875,-9.85223873629566));
#73333=CARTESIAN_POINT('Ctrl Pts',(-18.1410984204317,-20.9843249185812,
-9.85093631775104));
#73334=CARTESIAN_POINT('Ctrl Pts',(-18.1279527498485,-20.9804436402094,
-9.85012869961266));
#73335=CARTESIAN_POINT('Ctrl Pts',(-18.0291373443934,-20.9502218699535,
-9.84407038492819));
#73336=CARTESIAN_POINT('Ctrl Pts',(-17.9451747108148,-20.9185908271117,
-9.83899942898672));
#73337=CARTESIAN_POINT('Ctrl Pts',(-17.7339771197533,-20.823315479201,-9.82616914553694));
#73338=CARTESIAN_POINT('Ctrl Pts',(-17.6107065797325,-20.7520214298508,
-9.81861982055679));
#73339=CARTESIAN_POINT('Ctrl Pts',(-17.4517594198323,-20.6373657814144,
-9.80778302533903));
#73340=CARTESIAN_POINT('Ctrl Pts',(-17.4092366908299,-20.6041501435285,
-9.80475710136688));
#73341=CARTESIAN_POINT('Ctrl Pts',(-17.3466253420211,-20.5512703503387,
-9.80002727420146));
#73342=CARTESIAN_POINT('Ctrl Pts',(-17.3255811193627,-20.5327688572244,
-9.79838718134557));
#73343=CARTESIAN_POINT('Ctrl Pts',(-17.2998160340355,-20.5091939672304,
-9.79630625488515));
#73344=CARTESIAN_POINT('Ctrl Pts',(-17.2947435572111,-20.5045068723515,
-9.79589295518321));
#73345=CARTESIAN_POINT('Ctrl Pts',(-17.2867432949987,-20.4970415268961,
-9.79523516940728));
#73346=CARTESIAN_POINT('Ctrl Pts',(-17.2838003127209,-20.4942795325081,
-9.79499191100239));
#73347=CARTESIAN_POINT('Ctrl Pts',(-17.2782580721514,-20.4890482403505,
-9.79453133156171));
#73348=CARTESIAN_POINT('Ctrl Pts',(-17.2756571816422,-20.4865807496129,
-9.79431414798781));
#73349=CARTESIAN_POINT('Ctrl Pts',(-17.2697164939023,-20.4809160181113,
-9.79381570512716));
#73350=CARTESIAN_POINT('Ctrl Pts',(-17.266380897832,-20.4777144381185,-9.79353411174673));
#73351=CARTESIAN_POINT('Ctrl Pts',(-17.257535353891,-20.4691684387349,-9.79278282535843));
#73352=CARTESIAN_POINT('Ctrl Pts',(-17.2520439997879,-20.4638049914073,
-9.79231170494516));
#73353=CARTESIAN_POINT('Ctrl Pts',(-17.2132882755112,-20.425537927177,-9.78895388474047));
#73354=CARTESIAN_POINT('Ctrl Pts',(-17.1810961794957,-20.3915718693035,
-9.78599202321496));
#73355=CARTESIAN_POINT('Ctrl Pts',(-17.125316260505,-20.3286685569773,-9.78058303947507));
#73356=CARTESIAN_POINT('Ctrl Pts',(-17.1013166005308,-20.3001188335241,
-9.77815421222783));
#73357=CARTESIAN_POINT('Ctrl Pts',(-17.0034145093029,-20.1772048310218,
-9.76785133107912));
#73358=CARTESIAN_POINT('Ctrl Pts',(-16.9368360057211,-20.0772807742351,
-9.75986013238943));
#73359=CARTESIAN_POINT('Ctrl Pts',(-16.832227970176,-19.8870934150451,-9.7457418953503));
#73360=CARTESIAN_POINT('Ctrl Pts',(-16.7913005351884,-19.7987938478536,
-9.73956111761863));
#73361=CARTESIAN_POINT('Ctrl Pts',(-16.7488668865826,-19.6878004950989,
-9.73226044158712));
#73362=CARTESIAN_POINT('Ctrl Pts',(-16.741460351778,-19.667500979143,-9.73094324512345));
#73363=CARTESIAN_POINT('Ctrl Pts',(-16.7313955261904,-19.6385465398602,
-9.72908925942552));
#73364=CARTESIAN_POINT('Ctrl Pts',(-16.7284801478685,-19.6299830061242,
-9.72854397239901));
#73365=CARTESIAN_POINT('Ctrl Pts',(-16.7235539724407,-19.6152031739237,
-9.72760801752366));
#73366=CARTESIAN_POINT('Ctrl Pts',(-16.7215169142161,-19.6089958223235,
-9.72721648621118));
#73367=CARTESIAN_POINT('Ctrl Pts',(-16.7176772865902,-19.5971102270746,
-9.72646973591365));
#73368=CARTESIAN_POINT('Ctrl Pts',(-16.7158698908773,-19.5914336192741,
-9.72611436109393));
#73369=CARTESIAN_POINT('Ctrl Pts',(-16.7112444253581,-19.5766911355542,
-9.72519469576326));
#73370=CARTESIAN_POINT('Ctrl Pts',(-16.7084633142987,-19.5676137335427,
-9.72463162152827));
#73371=CARTESIAN_POINT('Ctrl Pts',(-16.6992477313659,-19.5367958958989,
-9.7227305302328));
#73372=CARTESIAN_POINT('Ctrl Pts',(-16.6931013323144,-19.5149704444151,
-9.721401902303));
#73373=CARTESIAN_POINT('Ctrl Pts',(-16.6414326919542,-19.3195173403618,
-9.70965054102293));
#73374=CARTESIAN_POINT('Ctrl Pts',(-16.6178134052955,-19.1408589724949,
-9.70001951991667));
#73375=CARTESIAN_POINT('Ctrl Pts',(-16.6166486753162,-18.8771219636983,
-9.68565936986543));
#73376=CARTESIAN_POINT('Ctrl Pts',(-16.6213037377898,-18.7929540282656,
-9.68103996703634));
#73377=CARTESIAN_POINT('Ctrl Pts',(-16.6352132691489,-18.6724279936042,
-9.6741078324025));
#73378=CARTESIAN_POINT('Ctrl Pts',(-16.6404363192971,-18.6356821462556,
-9.67195098004826));
#73379=CARTESIAN_POINT('Ctrl Pts',(-16.6478772898762,-18.5916699458051,
-9.66929497372547));
#73380=CARTESIAN_POINT('Ctrl Pts',(-16.6491722301562,-18.5842516133608,
-9.66884480030381));
#73381=CARTESIAN_POINT('Ctrl Pts',(-16.6512462681675,-18.5727331951739,
-9.66814170974775));
#73382=CARTESIAN_POINT('Ctrl Pts',(-16.651997972521,-18.5686281523267,-9.66789032309219));
#73383=CARTESIAN_POINT('Ctrl Pts',(-16.6534142251776,-18.5610210495021,
-9.66742292332395));
#73384=CARTESIAN_POINT('Ctrl Pts',(-16.6540754819808,-18.5575184353135,
-9.66720709886792));
#73385=CARTESIAN_POINT('Ctrl Pts',(-16.6555900121567,-18.549605791886,-9.66671815109773));
#73386=CARTESIAN_POINT('Ctrl Pts',(-16.6564484722836,-18.5451968226364,
-9.66644473670408));
#73387=CARTESIAN_POINT('Ctrl Pts',(-16.6590225197354,-18.5321974328358,
-9.66563580735149));
#73388=CARTESIAN_POINT('Ctrl Pts',(-16.6607773790297,-18.5236150133232,
-9.66509813241869));
#73389=CARTESIAN_POINT('Ctrl Pts',(-16.6738110976748,-18.4618279479156,
-9.66120246731753));
#73390=CARTESIAN_POINT('Ctrl Pts',(-16.6870823566694,-18.4090690423848,
-9.65774360085324));
#73391=CARTESIAN_POINT('Ctrl Pts',(-16.7108441930768,-18.3279498005957,
-9.65227698936044));
#73392=CARTESIAN_POINT('Ctrl Pts',(-16.7199369000747,-18.2992000357889,
-9.65030978437348));
#73393=CARTESIAN_POINT('Ctrl Pts',(-16.7713401227965,-18.1479835772066,
-9.63983436637738));
#73394=CARTESIAN_POINT('Ctrl Pts',(-16.824217386032,-18.0293894530551,-9.63119000482233));
#73395=CARTESIAN_POINT('Ctrl Pts',(-16.9306818126656,-17.8395766510796,
-9.61710026501743));
#73396=CARTESIAN_POINT('Ctrl Pts',(-16.978509845372,-17.7655347035796,-9.61152531949231));
#73397=CARTESIAN_POINT('Ctrl Pts',(-17.0429909979033,-17.6781877217658,
-9.60486247567757));
#73398=CARTESIAN_POINT('Ctrl Pts',(-17.0554042510384,-17.6618738343458,
-9.60361380607884));
#73399=CARTESIAN_POINT('Ctrl Pts',(-17.0735176763853,-17.6387727184145,
-9.60183895739354));
#73400=CARTESIAN_POINT('Ctrl Pts',(-17.079026259512,-17.6318373728369,-9.60130523435084));
#73401=CARTESIAN_POINT('Ctrl Pts',(-17.0886522634915,-17.619873105309,-9.6003828888715));
#73402=CARTESIAN_POINT('Ctrl Pts',(-17.0927495877286,-17.6148282371837,
-9.59999346825073));
#73403=CARTESIAN_POINT('Ctrl Pts',(-17.1006730807913,-17.6051636497448,
-9.59924643714513));
#73404=CARTESIAN_POINT('Ctrl Pts',(-17.1044957741889,-17.6005411739219,
-9.59888869152701));
#73405=CARTESIAN_POINT('Ctrl Pts',(-17.114563022773,-17.5884724735427,-9.59795344186742));
#73406=CARTESIAN_POINT('Ctrl Pts',(-17.120839340106,-17.5810528351643,-9.59737723875789));
#73407=CARTESIAN_POINT('Ctrl Pts',(-17.1428071232989,-17.5554430492663,
-9.59538384914218));
#73408=CARTESIAN_POINT('Ctrl Pts',(-17.1587573069793,-17.5374765414124,
-9.59397735247406));
#73409=CARTESIAN_POINT('Ctrl Pts',(-17.2748615069997,-17.4110952165873,
-9.58401517828428));
#73410=CARTESIAN_POINT('Ctrl Pts',(-17.3858071246414,-17.3131420658155,
-9.5759648193249));
#73411=CARTESIAN_POINT('Ctrl Pts',(-17.5440876299469,-17.2004356420584,
-9.56541234292053));
#73412=CARTESIAN_POINT('Ctrl Pts',(-17.5830075365717,-17.174618387826,-9.56287946376296));
#73413=CARTESIAN_POINT('Ctrl Pts',(-17.6835054484938,-17.1126399076543,
-9.55642055143619));
#73414=CARTESIAN_POINT('Ctrl Pts',(-17.7461140354447,-17.0782699973492,
-9.55247085455544));
#73415=CARTESIAN_POINT('Ctrl Pts',(-17.8405396986962,-17.0324832248759,
-9.54645231114514));
#73416=CARTESIAN_POINT('Ctrl Pts',(-17.871088305706,-17.0185577117792,-9.54449595810553));
#73417=CARTESIAN_POINT('Ctrl Pts',(-17.908675575444,-17.0024918458974,-9.54206250117054));
#73418=CARTESIAN_POINT('Ctrl Pts',(-17.9154128236215,-16.9996533402576,
-9.54162530516594));
#73419=CARTESIAN_POINT('Ctrl Pts',(-17.925974477908,-16.9952678328126,-9.54093814484613));
#73420=CARTESIAN_POINT('Ctrl Pts',(-17.9297890073633,-16.9936969853691,
-9.54068960116459));
#73421=CARTESIAN_POINT('Ctrl Pts',(-17.9369129055815,-16.9907876434509,
-9.5402247078457));
#73422=CARTESIAN_POINT('Ctrl Pts',(-17.9402210768033,-16.9894463665882,
-9.54000852936465));
#73423=CARTESIAN_POINT('Ctrl Pts',(-17.9477612673617,-16.9864114281703,
-9.5395151434047));
#73424=CARTESIAN_POINT('Ctrl Pts',(-17.9519953573566,-16.9847230707411,
-9.53923762199125));
#73425=CARTESIAN_POINT('Ctrl Pts',(-17.963017968391,-16.9803689753294,-9.53851399933805));
#73426=CARTESIAN_POINT('Ctrl Pts',(-17.9698148047226,-16.977724645775,-9.53806666262228));
#73427=CARTESIAN_POINT('Ctrl Pts',(-18.013179568873,-16.9611109354619,-9.53520602376663));
#73428=CARTESIAN_POINT('Ctrl Pts',(-18.0501129063736,-16.94812391682,-9.53274008093113));
#73429=CARTESIAN_POINT('Ctrl Pts',(-18.09913364696,-16.932399539207,-9.52944766422414));
#73430=CARTESIAN_POINT('Ctrl Pts',(-18.110917694779,-16.9287329050173,-9.52865473877205));
#73431=CARTESIAN_POINT('Ctrl Pts',(-18.1458489420505,-16.9181980711818,
-9.52630122535594));
#73432=CARTESIAN_POINT('Ctrl Pts',(-18.169081944689,-16.9116227110253,-9.52473195480415));
#73433=CARTESIAN_POINT('Ctrl Pts',(-18.3317801037737,-16.868567990221,-9.51373622242815));
#73434=CARTESIAN_POINT('Ctrl Pts',(-18.4745550596188,-16.8460172956255,
-9.50408909060972));
#73435=CARTESIAN_POINT('Ctrl Pts',(-18.6802311525133,-16.8347805084393,
-9.4907808297797));
#73436=CARTESIAN_POINT('Ctrl Pts',(-18.7420711537337,-16.8341129747927,
-9.48684923847594));
#73437=CARTESIAN_POINT('Ctrl Pts',(-18.841095182424,-16.8373823395173,-9.48067561603798));
#73438=CARTESIAN_POINT('Ctrl Pts',(-18.8782965828865,-16.8395947356132,
-9.47838366909235));
#73439=CARTESIAN_POINT('Ctrl Pts',(-18.9265161368928,-16.8437423012779,
-9.47544657393694));
#73440=CARTESIAN_POINT('Ctrl Pts',(-18.9376025871686,-16.8447840687048,
-9.47477359345177));
#73441=CARTESIAN_POINT('Ctrl Pts',(-18.9556144891969,-16.8466200821777,
-9.47368384270458));
#73442=CARTESIAN_POINT('Ctrl Pts',(-18.9625450384104,-16.8473611361049,
-9.47326540656282));
#73443=CARTESIAN_POINT('Ctrl Pts',(-18.975862700996,-16.8488516960841,-9.47246298271339));
#73444=CARTESIAN_POINT('Ctrl Pts',(-18.9822502967018,-16.8495961030302,
-9.47207883908743));
#73445=CARTESIAN_POINT('Ctrl Pts',(-18.9968632841322,-16.8513666189717,
-9.47120164581598));
#73446=CARTESIAN_POINT('Ctrl Pts',(-19.0050862730904,-16.8524119587024,
-9.47070920810994));
#73447=CARTESIAN_POINT('Ctrl Pts',(-19.0269054791241,-16.8553160263316,
-9.46940555241348));
#73448=CARTESIAN_POINT('Ctrl Pts',(-19.0404902642397,-16.8572587185303,
-9.46859698616855));
#73449=CARTESIAN_POINT('Ctrl Pts',(-19.1432878681387,-16.8729807320672,
-9.4625001512217));
#73450=CARTESIAN_POINT('Ctrl Pts',(-19.2315619322145,-16.8923221941895,
-9.45739437134887));
#73451=CARTESIAN_POINT('Ctrl Pts',(-19.4524106249719,-16.9557453951669,
-9.44467439946604));
#73452=CARTESIAN_POINT('Ctrl Pts',(-19.5823413464641,-17.0074020005798,
-9.43725493722378));
#73453=CARTESIAN_POINT('Ctrl Pts',(-19.7553603436323,-17.0968533118509,
-9.426496199625));
#73454=CARTESIAN_POINT('Ctrl Pts',(-19.8034593232911,-17.1241591722003,
-9.42339809171695));
#73455=CARTESIAN_POINT('Ctrl Pts',(-19.8746319587823,-17.1683354940968,
-9.41856620426507));
#73456=CARTESIAN_POINT('Ctrl Pts',(-19.8985260666795,-17.1838429947864,
-9.41689955795282));
#73457=CARTESIAN_POINT('Ctrl Pts',(-19.9278456865798,-17.2037237946812,
-9.41478893695049));
#73458=CARTESIAN_POINT('Ctrl Pts',(-19.9335733762604,-17.2076488526192,
-9.4143734448464));
#73459=CARTESIAN_POINT('Ctrl Pts',(-19.942606417804,-17.2139045241028,-9.41371296238759));
#73460=CARTESIAN_POINT('Ctrl Pts',(-19.9459246364139,-17.2162165942969,
-9.41346921690699));
#73461=CARTESIAN_POINT('Ctrl Pts',(-19.9521703939516,-17.2205951564529,
-9.4130082616476));
#73462=CARTESIAN_POINT('Ctrl Pts',(-19.9550993185081,-17.2226595781681,
-9.41279119251213));
#73463=CARTESIAN_POINT('Ctrl Pts',(-19.9617838673207,-17.2273965607995,
-9.4122937239963));
#73464=CARTESIAN_POINT('Ctrl Pts',(-19.9655360090366,-17.2300739548765,
-9.41201299520463));
#73465=CARTESIAN_POINT('Ctrl Pts',(-19.9754745422914,-17.2372148369655,
-9.41126550719833));
#73466=CARTESIAN_POINT('Ctrl Pts',(-19.9816455371486,-17.2416994988799,
-9.41079734288748));
#73467=CARTESIAN_POINT('Ctrl Pts',(-20.0247024892636,-17.2733474136382,
-9.40750321031105));
#73468=CARTESIAN_POINT('Ctrl Pts',(-20.0607197076459,-17.3016662306517,
-9.40460517835694));
#73469=CARTESIAN_POINT('Ctrl Pts',(-20.1245701891533,-17.3553106737324,
-9.39924373375802));
#73470=CARTESIAN_POINT('Ctrl Pts',(-20.1527029732708,-17.3802545042879,
-9.39679636136647));
#73471=CARTESIAN_POINT('Ctrl Pts',(-20.2758195000087,-17.4954148755112,
-9.38574623983081));
#73472=CARTESIAN_POINT('Ctrl Pts',(-20.3629793690467,-17.5935900853675,
-9.37700304687893));
#73473=CARTESIAN_POINT('Ctrl Pts',(-20.4927973318511,-17.7704210507134,
-9.36279858849358));
#73474=CARTESIAN_POINT('Ctrl Pts',(-20.5405828581872,-17.8448601402593,
-9.35720319140505));
#73475=CARTESIAN_POINT('Ctrl Pts',(-20.5935715947112,-17.9400196480767,
-9.3505186859072));
#73476=CARTESIAN_POINT('Ctrl Pts',(-20.603301284846,-17.9581068962629,-9.3492676328467));
#73477=CARTESIAN_POINT('Ctrl Pts',(-20.6168513917212,-17.9841992996234,
-9.34749002346898));
#73478=CARTESIAN_POINT('Ctrl Pts',(-20.6208868719261,-17.9920908921971,
-9.34695589092577));
#73479=CARTESIAN_POINT('Ctrl Pts',(-20.627795797468,-18.0058135858679,-9.34603306533409));
#73480=CARTESIAN_POINT('Ctrl Pts',(-20.6306921438653,-18.0116329622653,
-9.34564357180678));
#73481=CARTESIAN_POINT('Ctrl Pts',(-20.6362088783901,-18.0228464369602,
-9.34489655859997));
#73482=CARTESIAN_POINT('Ctrl Pts',(-20.6388332360733,-18.0282385023041,
-9.34453890303502));
#73483=CARTESIAN_POINT('Ctrl Pts',(-20.6456466878981,-18.0423900748048,
-9.34360423846161));
#73484=CARTESIAN_POINT('Ctrl Pts',(-20.6497985237955,-18.0511674426622,
-9.34302852718004));
#73485=CARTESIAN_POINT('Ctrl Pts',(-20.6639911324903,-18.0817138848473,
-9.34103855239193));
#73486=CARTESIAN_POINT('Ctrl Pts',(-20.6737226582474,-18.1036252174408,
-9.33963492933289));
#73487=CARTESIAN_POINT('Ctrl Pts',(-20.7429144525703,-18.2668347027014,
-9.32934406891176));
#73488=CARTESIAN_POINT('Ctrl Pts',(-20.7872440731791,-18.4140553991742,
-9.32100723458071));
#73489=CARTESIAN_POINT('Ctrl Pts',(-20.839087984038,-18.6927191816881,-9.30561471876861));
#73490=CARTESIAN_POINT('Ctrl Pts',(-20.8510398086686,-18.8225565564254,
-9.29857231214665));
#73491=CARTESIAN_POINT('Ctrl Pts',(-20.850998895741,-18.9559243732588,-9.29078133015851));
#73492=CARTESIAN_POINT('Ctrl Pts',(-20.8509902917105,-18.9591992920498,
-9.29058966769631));
#73493=CARTESIAN_POINT('Ctrl Pts',(-20.8508966134014,-18.9781329928378,
-9.28947949059534));
#73494=CARTESIAN_POINT('Ctrl Pts',(-20.8506454051252,-18.9937899720814,
-9.2885531605265));
#73495=CARTESIAN_POINT('Ctrl Pts',(-20.8500635606029,-19.0152256289942,
-9.28727185036972));
#73496=CARTESIAN_POINT('Ctrl Pts',(-20.8498828710246,-19.0210083110181,
-9.28692488681997));
#73497=CARTESIAN_POINT('Ctrl Pts',(-20.849558006434,-19.0301981503566,-9.28637131489791));
#73498=CARTESIAN_POINT('Ctrl Pts',(-20.8494292968978,-19.0336058744959,
-9.28616556645554));
#73499=CARTESIAN_POINT('Ctrl Pts',(-20.849146397906,-19.0406449432384,-9.2857395573068));
#73500=CARTESIAN_POINT('Ctrl Pts',(-20.8489910906245,-19.0442761959381,
-9.2855192323764));
#73501=CARTESIAN_POINT('Ctrl Pts',(-20.8485986126162,-19.0529306526134,
-9.28499281799852));
#73502=CARTESIAN_POINT('Ctrl Pts',(-20.8483528935365,-19.0579534308632,
-9.28468625368016));
#73503=CARTESIAN_POINT('Ctrl Pts',(-20.8474631286402,-19.0749035421436,
-9.28364827220232));
#73504=CARTESIAN_POINT('Ctrl Pts',(-20.8467360466117,-19.0868260325307,
-9.28291242752136));
#73505=CARTESIAN_POINT('Ctrl Pts',(-20.8368860011543,-19.2285882718191,
-9.2740997440102));
#73506=CARTESIAN_POINT('Ctrl Pts',(-20.8159089736642,-19.3573131149155,
-9.26548282185087));
#73507=CARTESIAN_POINT('Ctrl Pts',(-20.7661583380872,-19.5492103473173,
-9.25238287201765));
#73508=CARTESIAN_POINT('Ctrl Pts',(-20.7459070626398,-19.6142266721053,
-9.24789438225943));
#73509=CARTESIAN_POINT('Ctrl Pts',(-20.7225807271506,-19.6781099721152,
-9.24346982890923));
#73510=CARTESIAN_POINT('Origin',(-18.734,-18.952,0.));
#73511=CARTESIAN_POINT('',(-20.7225805821191,-19.6781103693095,-8.44448865465826));
#73512=CARTESIAN_POINT('',(-20.7225804318258,-19.6781107809139,-8.66553671816755));
#73513=CARTESIAN_POINT('',(-20.7225805821191,-19.6781103693095,0.));
#73514=CARTESIAN_POINT('',(-20.8509999986719,-18.9519250126714,-8.71094372102528));
#73515=CARTESIAN_POINT('Ctrl Pts',(-20.7225804318258,-19.6781107809139,
-8.66553671816755));
#73516=CARTESIAN_POINT('Ctrl Pts',(-20.756070039132,-19.5863936772582,-8.67195993448919));
#73517=CARTESIAN_POINT('Ctrl Pts',(-20.7832013384852,-19.4923954521791,
-8.67845479377976));
#73518=CARTESIAN_POINT('Ctrl Pts',(-20.8168871681233,-19.3356413520089,
-8.68892803045935));
#73519=CARTESIAN_POINT('Ctrl Pts',(-20.8273110801215,-19.2739462484318,
-8.69296405635655));
#73520=CARTESIAN_POINT('Ctrl Pts',(-20.8382409136492,-19.1855831091221,
-8.69860368086808));
#73521=CARTESIAN_POINT('Ctrl Pts',(-20.840999390498,-19.1592306791796,-8.70026812315789));
#73522=CARTESIAN_POINT('Ctrl Pts',(-20.8463154977908,-19.0972226537623,
-8.70414340561251));
#73523=CARTESIAN_POINT('Ctrl Pts',(-20.8484662904148,-19.0615396384699,
-8.70634153903778));
#73524=CARTESIAN_POINT('Ctrl Pts',(-20.8501018469652,-19.0146622935275,
-8.70918916109573));
#73525=CARTESIAN_POINT('Ctrl Pts',(-20.8504028282684,-19.0035040360996,
-8.70986402003792));
#73526=CARTESIAN_POINT('Ctrl Pts',(-20.8507477576586,-18.9854074805868,
-8.71095383259111));
#73527=CARTESIAN_POINT('Ctrl Pts',(-20.8508458710089,-18.9784705400062,
-8.71137047554056));
#73528=CARTESIAN_POINT('Ctrl Pts',(-20.8509497984663,-18.9672073924015,
-8.71204518351584));
#73529=CARTESIAN_POINT('Ctrl Pts',(-20.8509764542952,-18.96288147049,-8.71230389906779));
#73530=CARTESIAN_POINT('Ctrl Pts',(-20.8509965706215,-18.9563852094995,
-8.71269178471987));
#73531=CARTESIAN_POINT('Ctrl Pts',(-20.8509999537557,-18.954214932766,-8.71282126450749));
#73532=CARTESIAN_POINT('Ctrl Pts',(-20.8509999995291,-18.9520446497005,
-8.71295064004092));
#73533=CARTESIAN_POINT('Ctrl Pts',(-20.8509999986719,-18.9519250126714,
-8.71094372102528));
#73534=CARTESIAN_POINT('Ctrl Pts',(-20.8509972790728,-18.8751468230116,
-8.71553605185446));
#73535=CARTESIAN_POINT('Ctrl Pts',(-20.8468134450973,-18.79845405233,-8.72012838268364));
#73536=CARTESIAN_POINT('Ctrl Pts',(-20.8385019469856,-18.7223033410474,
-8.72472071351282));
#73537=CARTESIAN_POINT('Ctrl Pts',(-20.8301661890791,-18.6459303592906,
-8.72932644854445));
#73538=CARTESIAN_POINT('Ctrl Pts',(-20.817678733725,-18.5701030045679,-8.73393218357608));
#73539=CARTESIAN_POINT('Ctrl Pts',(-20.8011445449259,-18.4952698494918,
-8.73853791860771));
#73540=CARTESIAN_POINT('Ctrl Pts',(-20.7845848825983,-18.4203214021249,
-8.74315074950135));
#73541=CARTESIAN_POINT('Ctrl Pts',(-20.7639661648778,-18.3463705997999,
-8.74776358039499));
#73542=CARTESIAN_POINT('Ctrl Pts',(-20.7394430352797,-18.2738501402727,
-8.75237641128863));
#73543=CARTESIAN_POINT('Ctrl Pts',(-20.714852135364,-18.2011292685364,-8.75700198986252));
#73544=CARTESIAN_POINT('Ctrl Pts',(-20.6863354068384,-18.1298470190297,
-8.76162756843642));
#73545=CARTESIAN_POINT('Ctrl Pts',(-20.6540955877916,-18.0604160534513,
-8.76625314701031));
#73546=CARTESIAN_POINT('Ctrl Pts',(-20.6367568977577,-18.023075831747,-8.76874079971715));
#73547=CARTESIAN_POINT('Ctrl Pts',(-20.6183421527928,-17.9862706239728,
-8.771228452424));
#73548=CARTESIAN_POINT('Ctrl Pts',(-20.598888138009,-17.950061262994,-8.77371610513084));
#73549=CARTESIAN_POINT('Ctrl Pts',(-20.5645713376047,-17.886188102246,-8.77810431406174));
#73550=CARTESIAN_POINT('Ctrl Pts',(-20.526902233303,-17.8239553476819,-8.78249252299264));
#73551=CARTESIAN_POINT('Ctrl Pts',(-20.4860618340582,-17.7637372640545,
-8.78688073192354));
#73552=CARTESIAN_POINT('Ctrl Pts',(-20.4452820487373,-17.7036085540475,
-8.79126242802481));
#73553=CARTESIAN_POINT('Ctrl Pts',(-20.4013405804883,-17.6454889751325,
-8.79564412412608));
#73554=CARTESIAN_POINT('Ctrl Pts',(-20.3544642120278,-17.589728097061,-8.80002582022735));
#73555=CARTESIAN_POINT('Ctrl Pts',(-20.3076429270308,-17.5340327424588,
-8.80440236748699));
#73556=CARTESIAN_POINT('Ctrl Pts',(-20.2578939016347,-17.4806909501821,
-8.80877891474663));
#73557=CARTESIAN_POINT('Ctrl Pts',(-20.2054860875598,-17.4300217826401,
-8.81315546200628));
#73558=CARTESIAN_POINT('Ctrl Pts',(-20.1531115097589,-17.3793847487478,
-8.81752923372325));
#73559=CARTESIAN_POINT('Ctrl Pts',(-20.0980818347929,-17.3314173110765,
-8.82190300544023));
#73560=CARTESIAN_POINT('Ctrl Pts',(-20.0407040448442,-17.2864029481331,
-8.82627677715721));
#73561=CARTESIAN_POINT('Ctrl Pts',(-19.9833437151498,-17.2414022832115,
-8.83064921792076));
#73562=CARTESIAN_POINT('Ctrl Pts',(-19.9236370683466,-17.1993532065247,
-8.83502165868432));
#73563=CARTESIAN_POINT('Ctrl Pts',(-19.8619241653159,-17.1604989318182,
-8.83939409944787));
#73564=CARTESIAN_POINT('Ctrl Pts',(-19.8002096842795,-17.1216436636036,
-8.84376665201522));
#73565=CARTESIAN_POINT('Ctrl Pts',(-19.7364892544389,-17.0859836148755,
-8.84813920458256));
#73566=CARTESIAN_POINT('Ctrl Pts',(-19.6711304798855,-17.0537177597445,
-8.8525117571499));
#73567=CARTESIAN_POINT('Ctrl Pts',(-19.6057038735305,-17.0214184178919,
-8.85688884771723));
#73568=CARTESIAN_POINT('Ctrl Pts',(-19.5386359610935,-16.9925205167793,
-8.86126593828456));
#73569=CARTESIAN_POINT('Ctrl Pts',(-19.4703166749601,-16.9671758883529,
-8.86564302885189));
#73570=CARTESIAN_POINT('Ctrl Pts',(-19.4019600771288,-16.9418174182843,
-8.87002250991083));
#73571=CARTESIAN_POINT('Ctrl Pts',(-19.3323512055631,-16.9200162288386,
-8.87440199096978));
#73572=CARTESIAN_POINT('Ctrl Pts',(-19.2618949953266,-16.9018741809564,
-8.87878147202872));
#73573=CARTESIAN_POINT('Ctrl Pts',(-19.1913139019304,-16.8836999764162,
-8.88316871568844));
#73574=CARTESIAN_POINT('Ctrl Pts',(-19.1198829437759,-16.8691979613858,
-8.88755595934816));
#73575=CARTESIAN_POINT('Ctrl Pts',(-19.0480164983078,-16.858418704996,-8.89194320300788));
#73576=CARTESIAN_POINT('Ctrl Pts',(-18.9991542404241,-16.8510898493377,
-8.89492610594268));
#73577=CARTESIAN_POINT('Ctrl Pts',(-18.9500908178364,-16.8454808253817,
-8.89790900887748));
#73578=CARTESIAN_POINT('Ctrl Pts',(-18.900956661124,-16.8415937658104,-8.90089191181227));
#73579=CARTESIAN_POINT('Ctrl Pts',(-18.8286744078926,-16.8358754337365,
-8.90528012074316));
#73580=CARTESIAN_POINT('Ctrl Pts',(-18.7559569381437,-16.8338637794812,
-8.90966832967406));
#73581=CARTESIAN_POINT('Ctrl Pts',(-18.6832169260197,-16.8356091855716,
-8.91405653860495));
#73582=CARTESIAN_POINT('Ctrl Pts',(-18.6105848721342,-16.8373520011899,
-8.91843823470622));
#73583=CARTESIAN_POINT('Ctrl Pts',(-18.5379308205421,-16.8428407963575,
-8.92281993080749));
#73584=CARTESIAN_POINT('Ctrl Pts',(-18.4656714572672,-16.8520740981752,
-8.92720162690876));
#73585=CARTESIAN_POINT('Ctrl Pts',(-18.3934970044949,-16.8612965501284,
-8.9315781741684));
#73586=CARTESIAN_POINT('Ctrl Pts',(-18.3217167948298,-16.8742547070803,
-8.93595472142803));
#73587=CARTESIAN_POINT('Ctrl Pts',(-18.2507446877308,-16.8908951256271,
-8.94033126868767));
#73588=CARTESIAN_POINT('Ctrl Pts',(-18.1798175901105,-16.9075249910624,
-8.94470504040464));
#73589=CARTESIAN_POINT('Ctrl Pts',(-18.1096980467019,-16.9278323748368,
-8.94907881212161));
#73590=CARTESIAN_POINT('Ctrl Pts',(-18.0407905817006,-16.9517125950552,
-8.95345258383859));
#73591=CARTESIAN_POINT('Ctrl Pts',(-17.9719040854723,-16.9755855484423,
-8.95782502460214));
#73592=CARTESIAN_POINT('Ctrl Pts',(-17.9042293909009,-17.0030290219352,
-8.96219746536569));
#73593=CARTESIAN_POINT('Ctrl Pts',(-17.8381550707623,-17.0338887251363,
-8.96656990612925));
#73594=CARTESIAN_POINT('Ctrl Pts',(-17.7720790610961,-17.0647492174235,
-8.97094245869659));
#73595=CARTESIAN_POINT('Ctrl Pts',(-17.7076039433217,-17.0990259069124,
-8.97531501126393));
#73596=CARTESIAN_POINT('Ctrl Pts',(-17.6450960003002,-17.1365173976494,
-8.97968756383127));
#73597=CARTESIAN_POINT('Ctrl Pts',(-17.5825231841776,-17.1740477984696,
-8.98406465439859));
#73598=CARTESIAN_POINT('Ctrl Pts',(-17.5219220335754,-17.2147994133216,
-8.98844174496592));
#73599=CARTESIAN_POINT('Ctrl Pts',(-17.463631278137,-17.25852655453,-8.99281883553324));
#73600=CARTESIAN_POINT('Ctrl Pts',(-17.4053086879535,-17.3022775767532,
-8.99719831659219));
#73601=CARTESIAN_POINT('Ctrl Pts',(-17.3492993758008,-17.3490070515425,
-9.00157779765112));
#73602=CARTESIAN_POINT('Ctrl Pts',(-17.2959081742799,-17.3984296279868,
-9.00595727871007));
#73603=CARTESIAN_POINT('Ctrl Pts',(-17.2424223372128,-17.4479398056162,
-9.01034452236979));
#73604=CARTESIAN_POINT('Ctrl Pts',(-17.1915642147122,-17.5001522715464,
-9.01473176602951));
#73605=CARTESIAN_POINT('Ctrl Pts',(-17.1436006220657,-17.5547459720344,
-9.01911900968923));
#73606=CARTESIAN_POINT('Ctrl Pts',(-17.1109900008268,-17.5918644277299,
-9.02210191262405));
#73607=CARTESIAN_POINT('Ctrl Pts',(-17.0797165992414,-17.6300829433876,
-9.02508481555887));
#73608=CARTESIAN_POINT('Ctrl Pts',(-17.0498528101568,-17.6692930019123,
-9.0280677184937));
#73609=CARTESIAN_POINT('Ctrl Pts',(-17.0059195850955,-17.7269757132704,
-9.03245592742459));
#73610=CARTESIAN_POINT('Ctrl Pts',(-16.9648675150388,-17.7870307272458,
-9.03684413635549));
#73611=CARTESIAN_POINT('Ctrl Pts',(-16.926962336405,-17.8491383212981,-9.04123234528639));
#73612=CARTESIAN_POINT('Ctrl Pts',(-16.8891134153411,-17.9111537373832,
-9.04561404138765));
#73613=CARTESIAN_POINT('Ctrl Pts',(-16.8544023633227,-17.9752152777401,
-9.04999573748892));
#73614=CARTESIAN_POINT('Ctrl Pts',(-16.8230534861162,-18.0409717781125,
-9.05437743359019));
#73615=CARTESIAN_POINT('Ctrl Pts',(-16.7917414463353,-18.106651009364,-9.05875398084983));
#73616=CARTESIAN_POINT('Ctrl Pts',(-16.7637839395867,-18.174020810815,-9.06313052810946));
#73617=CARTESIAN_POINT('Ctrl Pts',(-16.739360042701,-18.2427042642548,-9.0675070753691));
#73618=CARTESIAN_POINT('Ctrl Pts',(-16.7149516350958,-18.3113441596467,
-9.07188084708608));
#73619=CARTESIAN_POINT('Ctrl Pts',(-16.6940725522121,-18.3812956006721,
-9.07625461880305));
#73620=CARTESIAN_POINT('Ctrl Pts',(-16.6768537344172,-18.4521617841754,
-9.08062839052003));
#73621=CARTESIAN_POINT('Ctrl Pts',(-16.6596401563663,-18.5230064028611,
-9.08500083128358));
#73622=CARTESIAN_POINT('Ctrl Pts',(-16.6460847459307,-18.5947647429381,
-9.08937327204712));
#73623=CARTESIAN_POINT('Ctrl Pts',(-16.6362680963765,-18.667026561729,-9.09374571281068));
#73624=CARTESIAN_POINT('Ctrl Pts',(-16.6264511958094,-18.7392902282626,
-9.09811826537802));
#73625=CARTESIAN_POINT('Ctrl Pts',(-16.620373308882,-18.8120569208139,-9.10249081794537));
#73626=CARTESIAN_POINT('Ctrl Pts',(-16.6180633554341,-18.8849096416521,
-9.10686337051271));
#73627=CARTESIAN_POINT('Ctrl Pts',(-16.6157510046294,-18.957837971792,-9.11124046108004));
#73628=CARTESIAN_POINT('Ctrl Pts',(-16.6172144102078,-19.0308520253124,
-9.11561755164736));
#73629=CARTESIAN_POINT('Ctrl Pts',(-16.6224303356467,-19.1035339981093,
-9.11999464221469));
#73630=CARTESIAN_POINT('Ctrl Pts',(-16.6276491096961,-19.1762556652293,
-9.12437412327363));
#73631=CARTESIAN_POINT('Ctrl Pts',(-16.6366244245266,-19.2486444114927,
-9.12875360433257));
#73632=CARTESIAN_POINT('Ctrl Pts',(-16.649281345285,-19.320289465887,-9.13313308539151));
#73633=CARTESIAN_POINT('Ctrl Pts',(-16.6619607003505,-19.3920615106593,
-9.13752032905123));
#73634=CARTESIAN_POINT('Ctrl Pts',(-16.6783345842869,-19.4630867607301,
-9.14190757271095));
#73635=CARTESIAN_POINT('Ctrl Pts',(-16.6982774637589,-19.5329670863655,
-9.14629481637068));
#73636=CARTESIAN_POINT('Ctrl Pts',(-16.7118367001085,-19.5804789741454,
-9.1492777193055));
#73637=CARTESIAN_POINT('Ctrl Pts',(-16.7270447244343,-19.6274619134097,
-9.15226062224032));
#73638=CARTESIAN_POINT('Ctrl Pts',(-16.7438494759073,-19.6737962949846,
-9.15524352517514));
#73639=CARTESIAN_POINT('Ctrl Pts',(-16.7685712862063,-19.7419597422966,
-9.15963173410604));
#73640=CARTESIAN_POINT('Ctrl Pts',(-16.7968473421401,-19.8089846766148,
-9.16401994303694));
#73641=CARTESIAN_POINT('Ctrl Pts',(-16.8285526457323,-19.8744745959181,
-9.16840815196783));
#73642=CARTESIAN_POINT('Ctrl Pts',(-16.8602108933972,-19.9398673173227,
-9.1727898480691));
#73643=CARTESIAN_POINT('Ctrl Pts',(-16.8952880767684,-20.0037291156991,
-9.17717154417037));
#73644=CARTESIAN_POINT('Ctrl Pts',(-16.9336103347365,-20.0656813068434,
-9.18155324027164));
#73645=CARTESIAN_POINT('Ctrl Pts',(-16.9718875610017,-20.1275606992327,
-9.18592978753128));
#73646=CARTESIAN_POINT('Ctrl Pts',(-17.0134020343728,-20.187534533793,-9.19030633479092));
#73647=CARTESIAN_POINT('Ctrl Pts',(-17.0579337571752,-20.2452482165706,
-9.19468288205056));
#73648=CARTESIAN_POINT('Ctrl Pts',(-17.1024372386062,-20.3029252981694,
-9.19905665376753));
#73649=CARTESIAN_POINT('Ctrl Pts',(-17.1499538788912,-20.3583446909812,
-9.20343042548451));
#73650=CARTESIAN_POINT('Ctrl Pts',(-17.2002209049092,-20.4111815128566,
-9.20780419720148));
#73651=CARTESIAN_POINT('Ctrl Pts',(-17.2504726345023,-20.4640022563097,
-9.21217663796503));
#73652=CARTESIAN_POINT('Ctrl Pts',(-17.3034727559334,-20.514241639775,-9.21654907872858));
#73653=CARTESIAN_POINT('Ctrl Pts',(-17.3589199436397,-20.5616098404893,
-9.22092151949214));
#73654=CARTESIAN_POINT('Ctrl Pts',(-17.4143685491366,-20.6089792524138,
-9.22529407205948));
#73655=CARTESIAN_POINT('Ctrl Pts',(-17.4722639770758,-20.6534770240218,
-9.22966662462682));
#73656=CARTESIAN_POINT('Ctrl Pts',(-17.5322712521182,-20.694853125342,-9.23403917719417));
#73657=CARTESIAN_POINT('Ctrl Pts',(-17.592340804974,-20.7362721683409,-9.23841626776149));
#73658=CARTESIAN_POINT('Ctrl Pts',(-17.6545261829441,-20.7745627981879,
-9.24279335832882));
#73659=CARTESIAN_POINT('Ctrl Pts',(-17.718463501407,-20.8095184036842,-9.24717044889615));
#73660=CARTESIAN_POINT('Ctrl Pts',(-17.7824357384127,-20.8444930997341,
-9.25154992995509));
#73661=CARTESIAN_POINT('Ctrl Pts',(-17.8481613859402,-20.8761289357272,
-9.25592941101403));
#73662=CARTESIAN_POINT('Ctrl Pts',(-17.9152544897592,-20.9042665774582,
-9.26030889207298));
#73663=CARTESIAN_POINT('Ctrl Pts',(-17.9824665156543,-20.9324540929703,
-9.2646961357327));
#73664=CARTESIAN_POINT('Ctrl Pts',(-18.051050383794,-20.9571308685661,-9.26908337939242));
#73665=CARTESIAN_POINT('Ctrl Pts',(-18.1206033812636,-20.9781869578404,
-9.27347062305214));
#73666=CARTESIAN_POINT('Ctrl Pts',(-18.1678927174319,-20.992503069587,-9.27645352598695));
#73667=CARTESIAN_POINT('Ctrl Pts',(-18.2156297492661,-21.0051465017728,
-9.27943642892176));
#73668=CARTESIAN_POINT('Ctrl Pts',(-18.2636857248405,-21.0160962871391,
-9.28241933185657));
#73669=CARTESIAN_POINT('Ctrl Pts',(-18.3343818439592,-21.0322047381968,
-9.28680754078746));
#73670=CARTESIAN_POINT('Ctrl Pts',(-18.4060444995741,-21.0447083756574,
-9.29119574971836));
#73671=CARTESIAN_POINT('Ctrl Pts',(-18.4782726371996,-21.0534976840137,
-9.29558395864926));
#73672=CARTESIAN_POINT('Ctrl Pts',(-18.5503935762932,-21.0622739475792,
-9.29996565475053));
#73673=CARTESIAN_POINT('Ctrl Pts',(-18.6230778564465,-21.0673467676749,
-9.3043473508518));
#73674=CARTESIAN_POINT('Ctrl Pts',(-18.695912956451,-21.0686573594027,-9.30872904695307));
#73675=CARTESIAN_POINT('Ctrl Pts',(-18.7686624694166,-21.0699664110809,
-9.31310559421271));
#73676=CARTESIAN_POINT('Ctrl Pts',(-18.8415619702683,-21.0675220079374,
-9.31748214147234));
#73677=CARTESIAN_POINT('Ctrl Pts',(-18.9141942210379,-21.0613171982195,
-9.32185868873198));
#73678=CARTESIAN_POINT('Ctrl Pts',(-18.9867804094897,-21.0551163235017,
-9.32623246044896));
#73679=CARTESIAN_POINT('Ctrl Pts',(-19.0590992046973,-21.0451598149104,
-9.33060623216593));
#73680=CARTESIAN_POINT('Ctrl Pts',(-19.1307351980801,-21.0314927705102,
-9.3349800038829));
#73681=CARTESIAN_POINT('Ctrl Pts',(-19.2023493923896,-21.0178298850376,
-9.33935244464645));
#73682=CARTESIAN_POINT('Ctrl Pts',(-19.273280723833,-21.0004587957695,-9.34372488541001));
#73683=CARTESIAN_POINT('Ctrl Pts',(-19.3431223955197,-20.979475994254,-9.34809732617356));
#73684=CARTESIAN_POINT('Ctrl Pts',(-19.4129658530657,-20.9584926562059,
-9.35246987874091));
#73685=CARTESIAN_POINT('Ctrl Pts',(-19.4817191341329,-20.9338975632636,
-9.35684243130824));
#73686=CARTESIAN_POINT('Ctrl Pts',(-19.5489906872856,-20.9058370401949,
-9.36121498387559));
#73687=CARTESIAN_POINT('Ctrl Pts',(-19.6163320573937,-20.877747394857,-9.36559207444291));
#73688=CARTESIAN_POINT('Ctrl Pts',(-19.6821881831277,-20.8461853247306,
-9.36996916501024));
#73689=CARTESIAN_POINT('Ctrl Pts',(-19.7461883733224,-20.8113449644729,
-9.37434625557757));
#73690=CARTESIAN_POINT('Ctrl Pts',(-19.8102235163964,-20.7764855766014,
-9.37872573663651));
#73691=CARTESIAN_POINT('Ctrl Pts',(-19.8724002944082,-20.738344586342,-9.38310521769545));
#73692=CARTESIAN_POINT('Ctrl Pts',(-19.9323758228015,-20.6971602755406,
-9.38748469875439));
#73693=CARTESIAN_POINT('Ctrl Pts',(-19.9924576574162,-20.6559029658247,
-9.39187194241411));
#73694=CARTESIAN_POINT('Ctrl Pts',(-20.0503300675359,-20.6115918569496,
-9.39625918607383));
#73695=CARTESIAN_POINT('Ctrl Pts',(-20.1056826247706,-20.5645060548421,
-9.40064642973355));
#73696=CARTESIAN_POINT('Ctrl Pts',(-20.1433170299305,-20.532492246586,-9.40362933266837));
#73697=CARTESIAN_POINT('Ctrl Pts',(-20.1797873054598,-20.4991966074029,
-9.40661223560319));
#73698=CARTESIAN_POINT('Ctrl Pts',(-20.2150061302366,-20.4647160481074,
-9.409595138538));
#73699=CARTESIAN_POINT('Ctrl Pts',(-20.2660736595598,-20.4147190086245,
-9.41392036756134));
#73700=CARTESIAN_POINT('Ctrl Pts',(-20.3147200093879,-20.3620217118595,
-9.41824559658467));
#73701=CARTESIAN_POINT('Ctrl Pts',(-20.3606400168238,-20.3068916029216,
-9.422570825608));
#73702=CARTESIAN_POINT('Ctrl Pts',(-20.4064831242461,-20.2518538177085,
-9.42688881137966));
#73703=CARTESIAN_POINT('Ctrl Pts',(-20.4496086381081,-20.194391687308,-9.43120679715132));
#73704=CARTESIAN_POINT('Ctrl Pts',(-20.4897475359155,-20.1348100397472,
-9.43552478292298));
#73705=CARTESIAN_POINT('Ctrl Pts',(-20.5298476914605,-20.0752859006867,
-9.43983860095346));
#73706=CARTESIAN_POINT('Ctrl Pts',(-20.5669666687588,-20.0136467099182,
-9.44415241898393));
#73707=CARTESIAN_POINT('Ctrl Pts',(-20.6008760498832,-19.9502298404538,
-9.44846623701441));
#73708=CARTESIAN_POINT('Ctrl Pts',(-20.634764851022,-19.8868514594022,-9.4527774369401));
#73709=CARTESIAN_POINT('Ctrl Pts',(-20.6654476851597,-19.8216979770398,
-9.45708863686578));
#73710=CARTESIAN_POINT('Ctrl Pts',(-20.6927407815271,-19.7551335821535,
-9.46139983679147));
#73711=CARTESIAN_POINT('Ctrl Pts',(-20.7031862176723,-19.7296584903219,
-9.4630497911582));
#73712=CARTESIAN_POINT('Ctrl Pts',(-20.7131356416779,-19.7039769950381,
-9.46469974552493));
#73713=CARTESIAN_POINT('Ctrl Pts',(-20.7225805821191,-19.6781103693095,
-9.46634969989166));
#73714=CARTESIAN_POINT('',(-20.8509991049198,-18.9500532671891,-8.48905627902251));
#73715=CARTESIAN_POINT('Ctrl Pts',(-20.7225807271506,-19.6781099721152,
-9.24346982890923));
#73716=CARTESIAN_POINT('Ctrl Pts',(-20.6903081412074,-19.7664941630596,
-9.23734834539027));
#73717=CARTESIAN_POINT('Ctrl Pts',(-20.6521492195846,-19.8527097500488,
-9.23135288011962));
#73718=CARTESIAN_POINT('Ctrl Pts',(-20.5973011252839,-19.9571668947513,
-9.22408573268242));
#73719=CARTESIAN_POINT('Ctrl Pts',(-20.5859221923446,-19.9779804262763,
-9.22263712070413));
#73720=CARTESIAN_POINT('Ctrl Pts',(-20.5694164036234,-20.0070019308189,
-9.22061563734104));
#73721=CARTESIAN_POINT('Ctrl Pts',(-20.5645797432616,-20.015372116021,-9.22003242009133));
#73722=CARTESIAN_POINT('Ctrl Pts',(-20.5566540595066,-20.0288737371604,
-9.21909125274794));
#73723=CARTESIAN_POINT('Ctrl Pts',(-20.5536003367204,-20.0340256384089,
-9.21873202952226));
#73724=CARTESIAN_POINT('Ctrl Pts',(-20.5471835377953,-20.0447473586356,
-9.21798421248231));
#73725=CARTESIAN_POINT('Ctrl Pts',(-20.5438165598497,-20.0503147785078,
-9.21759576604661));
#73726=CARTESIAN_POINT('Ctrl Pts',(-20.5357843430347,-20.0634591097778,
-9.21667830923621));
#73727=CARTESIAN_POINT('Ctrl Pts',(-20.5310968725028,-20.0710223438505,
-9.21615012147147));
#73728=CARTESIAN_POINT('Ctrl Pts',(-20.5153273240207,-20.0961118548183,
-9.21439682040229));
#73729=CARTESIAN_POINT('Ctrl Pts',(-20.5040352295017,-20.1135051885399,
-9.21317948307665));
#73730=CARTESIAN_POINT('Ctrl Pts',(-20.442391950146,-20.205467732651,-9.20672839923418));
#73731=CARTESIAN_POINT('Ctrl Pts',(-20.3875781975563,-20.2769400880788,
-9.20166760661514));
#73732=CARTESIAN_POINT('Ctrl Pts',(-20.239228168277,-20.4467709831743,-9.18923032568631));
#73733=CARTESIAN_POINT('Ctrl Pts',(-20.14049106098,-20.5400279545725,-9.18201783936024));
#73734=CARTESIAN_POINT('Ctrl Pts',(-19.9740096098071,-20.6694831918039,
-9.17034208316701));
#73735=CARTESIAN_POINT('Ctrl Pts',(-19.9120736714761,-20.7125431584589,
-9.16608185049325));
#73736=CARTESIAN_POINT('Ctrl Pts',(-19.8399119400585,-20.757197449934,-9.16105241312598));
#73737=CARTESIAN_POINT('Ctrl Pts',(-19.8318090901944,-20.7621365269822,
-9.16048676398966));
#73738=CARTESIAN_POINT('Ctrl Pts',(-19.819747292292,-20.7693779982016,-9.15964298569349));
#73739=CARTESIAN_POINT('Ctrl Pts',(-19.8158135092527,-20.7717223693083,
-9.15936752405193));
#73740=CARTESIAN_POINT('Ctrl Pts',(-19.8087980895348,-20.7758724801802,
-9.1588757258892));
#73741=CARTESIAN_POINT('Ctrl Pts',(-19.805719459314,-20.777683202947,-9.15865971786735));
#73742=CARTESIAN_POINT('Ctrl Pts',(-19.7990873449481,-20.7815613815112,
-9.15819396370905));
#73743=CARTESIAN_POINT('Ctrl Pts',(-19.7955324686047,-20.7836262496808,
-9.15794406161423));
#73744=CARTESIAN_POINT('Ctrl Pts',(-19.7856954071848,-20.78930190073,-9.15725188192812));
#73745=CARTESIAN_POINT('Ctrl Pts',(-19.7794007327574,-20.7928907649215,
-9.15680823068811));
#73746=CARTESIAN_POINT('Ctrl Pts',(-19.7446837696283,-20.8124489151308,
-9.15435789212968));
#73747=CARTESIAN_POINT('Ctrl Pts',(-19.7159155890041,-20.8277913938971,
-9.15231471694279));
#73748=CARTESIAN_POINT('Ctrl Pts',(-19.5415625181828,-20.9156665823046,
-9.13990730862574));
#73749=CARTESIAN_POINT('Ctrl Pts',(-19.3883704470067,-20.9718868591919,
-9.12895421470627));
#73750=CARTESIAN_POINT('Ctrl Pts',(-19.1167158273123,-21.0373915602516,
-9.1107014580258));
#73751=CARTESIAN_POINT('Ctrl Pts',(-19.0010932404552,-21.0553303039268,
-9.10326192697726));
#73752=CARTESIAN_POINT('Ctrl Pts',(-18.8703108117004,-21.0646553293364,
-9.09525608838018));
#73753=CARTESIAN_POINT('Ctrl Pts',(-18.8560477217907,-21.0655272762096,
-9.09438812835139));
#73754=CARTESIAN_POINT('Ctrl Pts',(-18.8333331427384,-21.0666851785229,
-9.09301384026215));
#73755=CARTESIAN_POINT('Ctrl Pts',(-18.8248870723574,-21.067065015745,-9.09250458426938));
#73756=CARTESIAN_POINT('Ctrl Pts',(-18.8099870479676,-21.0676456833767,
-9.09160921151416));
#73757=CARTESIAN_POINT('Ctrl Pts',(-18.803534068515,-21.067867600725,-9.09122243864934));
#73758=CARTESIAN_POINT('Ctrl Pts',(-18.7901850938562,-21.0682655359961,
-9.09042436892466));
#73759=CARTESIAN_POINT('Ctrl Pts',(-18.7832890437421,-21.0684373781228,
-9.09001320745828));
#73760=CARTESIAN_POINT('Ctrl Pts',(-18.7655855916307,-21.068791954899,-9.08896048784528));
#73761=CARTESIAN_POINT('Ctrl Pts',(-18.7547773227515,-21.0689256338714,
-9.08832047105696));
#73762=CARTESIAN_POINT('Ctrl Pts',(-18.7096624019784,-21.0691380695378,
-9.0856597279634));
#73763=CARTESIAN_POINT('Ctrl Pts',(-18.6753562818806,-21.0684656942907,
-9.08366253215187));
#73764=CARTESIAN_POINT('Ctrl Pts',(-18.5860256197608,-21.0645409901289,
-9.07851824069386));
#73765=CARTESIAN_POINT('Ctrl Pts',(-18.5310840268167,-21.0599733407905,
-9.07541053833727));
#73766=CARTESIAN_POINT('Ctrl Pts',(-18.3678442175265,-21.0399597833096,
-9.066265877723));
#73767=CARTESIAN_POINT('Ctrl Pts',(-18.260499454246,-21.0182633496938,-9.06037764802157));
#73768=CARTESIAN_POINT('Ctrl Pts',(-18.1111162202479,-20.9758121872233,
-9.0519225662748));
#73769=CARTESIAN_POINT('Ctrl Pts',(-18.0673425814505,-20.9618178069699,
-9.04941031793161));
#73770=CARTESIAN_POINT('Ctrl Pts',(-18.00306649288,-20.9389377932736,-9.04562658902648));
#73771=CARTESIAN_POINT('Ctrl Pts',(-17.982192497875,-20.9311339059033,-9.04438257031487));
#73772=CARTESIAN_POINT('Ctrl Pts',(-17.9135890799748,-20.9042441144118,
-9.04023182440806));
#73773=CARTESIAN_POINT('Ctrl Pts',(-17.8664351868196,-20.8837508983648,
-9.03727821380553));
#73774=CARTESIAN_POINT('Ctrl Pts',(-17.8129725138501,-20.8581635350126,
-9.03376034207724));
#73775=CARTESIAN_POINT('Ctrl Pts',(-17.8058862038966,-20.8547232666823,
-9.03329055270424));
#73776=CARTESIAN_POINT('Ctrl Pts',(-17.7946186247985,-20.8491751518349,
-9.03253770002197));
#73777=CARTESIAN_POINT('Ctrl Pts',(-17.790424785836,-20.8470928048693,-9.03225618189817));
#73778=CARTESIAN_POINT('Ctrl Pts',(-17.7830250350207,-20.8433879893595,
-9.03175709443563));
#73779=CARTESIAN_POINT('Ctrl Pts',(-17.7798163024653,-20.8417712511085,
-9.03153988503455));
#73780=CARTESIAN_POINT('Ctrl Pts',(-17.7730412366998,-20.8383359405492,
-9.03107956131357));
#73781=CARTESIAN_POINT('Ctrl Pts',(-17.7694759969734,-20.8365154476262,
-9.03083633212184));
#73782=CARTESIAN_POINT('Ctrl Pts',(-17.7599055900177,-20.8315943064334,
-9.03018078606027));
#73783=CARTESIAN_POINT('Ctrl Pts',(-17.7539101309969,-20.8284750257231,
-9.02976732134429));
#73784=CARTESIAN_POINT('Ctrl Pts',(-17.7247066666117,-20.813103089231,-9.02774007496838));
#73785=CARTESIAN_POINT('Ctrl Pts',(-17.7017140521055,-20.8004488948402,
-9.02610285112236));
#73786=CARTESIAN_POINT('Ctrl Pts',(-17.6365300270785,-20.7629788185537,
-9.02135508998252));
#73787=CARTESIAN_POINT('Ctrl Pts',(-17.5949575681654,-20.7371236171926,
-9.01819698633989));
#73788=CARTESIAN_POINT('Ctrl Pts',(-17.4740669076194,-20.6559950283415,
-9.0086965865316));
#73789=CARTESIAN_POINT('Ctrl Pts',(-17.3975959971134,-20.5967050176867,
-9.00226746872186));
#73790=CARTESIAN_POINT('Ctrl Pts',(-17.220170089257,-20.4385712648393,-8.98663161768537));
#73791=CARTESIAN_POINT('Ctrl Pts',(-17.1245183702649,-20.3344461504433,
-8.97756396724562));
#73792=CARTESIAN_POINT('Ctrl Pts',(-17.0313564409232,-20.210132703032,-8.96807851641956));
#73793=CARTESIAN_POINT('Ctrl Pts',(-17.0229070111065,-20.1986169366562,
-8.96721096632442));
#73794=CARTESIAN_POINT('Ctrl Pts',(-17.0096435758668,-20.1801511989274,
-8.96583720257601));
#73795=CARTESIAN_POINT('Ctrl Pts',(-17.0047536536433,-20.1732565339541,
-8.96532806446533));
#73796=CARTESIAN_POINT('Ctrl Pts',(-16.9962016494398,-20.1610440760181,
-8.96443282881721));
#73797=CARTESIAN_POINT('Ctrl Pts',(-16.9925223806488,-20.1557385046993,
-8.96404607580978));
#73798=CARTESIAN_POINT('Ctrl Pts',(-16.9849620146775,-20.1447291060193,
-8.96324797986233));
#73799=CARTESIAN_POINT('Ctrl Pts',(-16.9810844076774,-20.1390229662357,
-8.96283677264725));
#73800=CARTESIAN_POINT('Ctrl Pts',(-16.9712013673956,-20.1243254190353,
-8.96178379676295));
#73801=CARTESIAN_POINT('Ctrl Pts',(-16.9652367522292,-20.1153067038098,
-8.9611435709255));
#73802=CARTESIAN_POINT('Ctrl Pts',(-16.9406197447854,-20.0774578275874,
-8.9584807951637));
#73803=CARTESIAN_POINT('Ctrl Pts',(-16.9226004577457,-20.0482207610384,
-8.95648182164581));
#73804=CARTESIAN_POINT('Ctrl Pts',(-16.8775013535254,-19.9708946076262,
-8.95133191531324));
#73805=CARTESIAN_POINT('Ctrl Pts',(-16.8515758316577,-19.9221615039678,
-8.94822048865645));
#73806=CARTESIAN_POINT('Ctrl Pts',(-16.7800131968833,-19.7739453648798,
-8.93906933130394));
#73807=CARTESIAN_POINT('Ctrl Pts',(-16.7401515465627,-19.6718804283087,
-8.93317830736694));
#73808=CARTESIAN_POINT('Ctrl Pts',(-16.6935615489729,-19.5184736083894,
-8.9244492072757));
#73809=CARTESIAN_POINT('Ctrl Pts',(-16.6805284935058,-19.4692386718673,
-8.92166384483347));
#73810=CARTESIAN_POINT('Ctrl Pts',(-16.6658125615088,-19.4042572979707,
-8.91795697512142));
#73811=CARTESIAN_POINT('Ctrl Pts',(-16.6625125134373,-19.38889303031,-8.91707827504095));
#73812=CARTESIAN_POINT('Ctrl Pts',(-16.648882110064,-19.3218034087935,-8.91322623530355));
#73813=CARTESIAN_POINT('Ctrl Pts',(-16.6403167669215,-19.2697431464976,
-8.91019828482176));
#73814=CARTESIAN_POINT('Ctrl Pts',(-16.6326149764804,-19.2087986341417,
-8.90655268787263));
#73815=CARTESIAN_POINT('Ctrl Pts',(-16.6315783128396,-19.2001684892654,
-8.90603410192148));
#73816=CARTESIAN_POINT('Ctrl Pts',(-16.630088263151,-19.1870839188921,-8.90524396788583));
#73817=CARTESIAN_POINT('Ctrl Pts',(-16.6295957989297,-19.1826339156402,
-8.90497456762527));
#73818=CARTESIAN_POINT('Ctrl Pts',(-16.6287367225723,-19.1746392415219,
-8.90448930231885));
#73819=CARTESIAN_POINT('Ctrl Pts',(-16.62836494123,-19.1710951805231,-8.90427373132515));
#73820=CARTESIAN_POINT('Ctrl Pts',(-16.6275760433204,-19.1633873812406,
-8.90380390383939));
#73821=CARTESIAN_POINT('Ctrl Pts',(-16.6271623283961,-19.1592233940286,
-8.9035494644057));
#73822=CARTESIAN_POINT('Ctrl Pts',(-16.6260337076674,-19.1475111210151,
-8.9028320861379));
#73823=CARTESIAN_POINT('Ctrl Pts',(-16.6253470127124,-19.1399602704302,
-8.90236760815954));
#73824=CARTESIAN_POINT('Ctrl Pts',(-16.6214621608634,-19.0945387584654,
-8.89956229864038));
#73825=CARTESIAN_POINT('Ctrl Pts',(-16.619243951302,-19.0565937786277,-8.89717171253788));
#73826=CARTESIAN_POINT('Ctrl Pts',(-16.6152879480915,-18.9309310782332,
-8.8891435145921));
#73827=CARTESIAN_POINT('Ctrl Pts',(-16.6179805379353,-18.8431682047451,
-8.88336091591602));
#73828=CARTESIAN_POINT('Ctrl Pts',(-16.6422708849619,-18.5821605699798,
-8.86604056163588));
#73829=CARTESIAN_POINT('Ctrl Pts',(-16.6798383381421,-18.4111166343265,
-8.85459340835551));
#73830=CARTESIAN_POINT('Ctrl Pts',(-16.745664606849,-18.2248525605343,-8.8424327332812));
#73831=CARTESIAN_POINT('Ctrl Pts',(-16.7537054639037,-18.2032312434783,
-8.84102457385064));
#73832=CARTESIAN_POINT('Ctrl Pts',(-16.7655761001365,-18.1728416630186,
-8.83904954357946));
#73833=CARTESIAN_POINT('Ctrl Pts',(-16.7691141688392,-18.1639619052149,
-8.83847295299369));
#73834=CARTESIAN_POINT('Ctrl Pts',(-16.7749592015262,-18.1495763093885,
-8.83753959559214));
#73835=CARTESIAN_POINT('Ctrl Pts',(-16.7772294957275,-18.1440558038561,
-8.83718159657123));
#73836=CARTESIAN_POINT('Ctrl Pts',(-16.7820294176574,-18.1325231000204,
-8.83643405809275));
#73837=CARTESIAN_POINT('Ctrl Pts',(-16.7845635470042,-18.1265128340607,
-8.83604467598862));
#73838=CARTESIAN_POINT('Ctrl Pts',(-16.7906560126747,-18.1122476858005,
-8.83512091297652));
#73839=CARTESIAN_POINT('Ctrl Pts',(-16.7942392461985,-18.1040035235427,
-8.83458738615579));
#73840=CARTESIAN_POINT('Ctrl Pts',(-16.8064770433044,-18.0763307636169,
-8.83279745971867));
#73841=CARTESIAN_POINT('Ctrl Pts',(-16.8153720280101,-18.057009433696,-8.83154929582967));
#73842=CARTESIAN_POINT('Ctrl Pts',(-16.8912564925192,-17.8985090925484,
-8.82131530963366));
#73843=CARTESIAN_POINT('Ctrl Pts',(-16.9730030260183,-17.7669076653599,
-8.81289798811847));
#73844=CARTESIAN_POINT('Ctrl Pts',(-17.1527697460017,-17.5377487914963,
-8.79708128694917));
#73845=CARTESIAN_POINT('Ctrl Pts',(-17.2474057534722,-17.4385857273095,
-8.78969570626167));
#73846=CARTESIAN_POINT('Ctrl Pts',(-17.3627250874046,-17.3390719013255,
-8.78076352063304));
#73847=CARTESIAN_POINT('Ctrl Pts',(-17.3746370382221,-17.3290199497087,
-8.77984141466584));
#73848=CARTESIAN_POINT('Ctrl Pts',(-17.3911125568151,-17.3154256325307,
-8.77856506099069));
#73849=CARTESIAN_POINT('Ctrl Pts',(-17.3955815749362,-17.3117687775827,
-8.77821875001981));
#73850=CARTESIAN_POINT('Ctrl Pts',(-17.4027117950377,-17.3059828889375,
-8.77766596222476));
#73851=CARTESIAN_POINT('Ctrl Pts',(-17.4053633114003,-17.3038418874666,
-8.77746034097041));
#73852=CARTESIAN_POINT('Ctrl Pts',(-17.410854392957,-17.2994299037098,-8.77703437292913));
#73853=CARTESIAN_POINT('Ctrl Pts',(-17.4136946347415,-17.2971598378449,
-8.77681396092256));
#73854=CARTESIAN_POINT('Ctrl Pts',(-17.4204832512033,-17.2917626315522,
-8.77628697249191));
#73855=CARTESIAN_POINT('Ctrl Pts',(-17.4244369532535,-17.2886422530457,
-8.77597991846356));
#73856=CARTESIAN_POINT('Ctrl Pts',(-17.4378410971752,-17.2781407192771,
-8.77493857470123));
#73857=CARTESIAN_POINT('Ctrl Pts',(-17.447342904198,-17.2708259175234,-8.77419981912154));
#73858=CARTESIAN_POINT('Ctrl Pts',(-17.5586182815263,-17.1866583801352,
-8.76554663027551));
#73859=CARTESIAN_POINT('Ctrl Pts',(-17.6670638480853,-17.119080546469,-8.75711321429331));
#73860=CARTESIAN_POINT('Ctrl Pts',(-17.9283007809298,-16.987367211882,-8.73777944961678));
#73861=CARTESIAN_POINT('Ctrl Pts',(-18.0838982063598,-16.9305350451299,
-8.726984085091));
#73862=CARTESIAN_POINT('Ctrl Pts',(-18.2675084998527,-16.8869014756195,
-8.71536079879259));
#73863=CARTESIAN_POINT('Ctrl Pts',(-18.2905651075062,-16.8818280742839,
-8.71391917588496));
#73864=CARTESIAN_POINT('Ctrl Pts',(-18.3231584781354,-16.875225739675,-8.71190572463697));
#73865=CARTESIAN_POINT('Ctrl Pts',(-18.3326275547124,-16.8733749136939,
-8.71132365980457));
#73866=CARTESIAN_POINT('Ctrl Pts',(-18.3479910214154,-16.8704808688451,
-8.71038385170174));
#73867=CARTESIAN_POINT('Ctrl Pts',(-18.3538776840689,-16.8693978173961,
-8.71002484244759));
#73868=CARTESIAN_POINT('Ctrl Pts',(-18.3661754091762,-16.8671891122747,
-8.70927708055056));
#73869=CARTESIAN_POINT('Ctrl Pts',(-18.3725872370408,-16.8660680300109,
-8.70888847699872));
#73870=CARTESIAN_POINT('Ctrl Pts',(-18.3877913035338,-16.863481868435,-8.7079699506935));
#73871=CARTESIAN_POINT('Ctrl Pts',(-18.3965878700561,-16.8620427024331,
-8.70744085588123));
#73872=CARTESIAN_POINT('Ctrl Pts',(-18.425380879748,-16.8575185361226,-8.70571644959349));
#73873=CARTESIAN_POINT('Ctrl Pts',(-18.4454128747005,-16.854664576923,-8.70452844975692));
#73874=CARTESIAN_POINT('Ctrl Pts',(-18.4930786997523,-16.8485694952434,
-8.70172743216196));
#73875=CARTESIAN_POINT('Ctrl Pts',(-18.5207418760511,-16.8455850280324,
-8.70012237341828));
#73876=CARTESIAN_POINT('Ctrl Pts',(-18.7171642363187,-16.8283032017231,
-8.68885173277689));
#73877=CARTESIAN_POINT('Ctrl Pts',(-18.8870379552048,-16.8337569676413,
-8.67982457081734));
#73878=CARTESIAN_POINT('Ctrl Pts',(-19.157209368514,-16.8751299374255,-8.66488771521993));
#73879=CARTESIAN_POINT('Ctrl Pts',(-19.2586536417649,-16.89841091196,-8.65912337343936));
#73880=CARTESIAN_POINT('Ctrl Pts',(-19.367220372226,-16.9318973257694,-8.65239234173926));
#73881=CARTESIAN_POINT('Ctrl Pts',(-19.3764579481692,-16.934816163307,-8.65181502958846));
#73882=CARTESIAN_POINT('Ctrl Pts',(-19.3900688512375,-16.939219835748,-8.65095716118084));
#73883=CARTESIAN_POINT('Ctrl Pts',(-19.3944580255002,-16.9406557920643,
-8.65067940341618));
#73884=CARTESIAN_POINT('Ctrl Pts',(-19.4022370968834,-16.9432289908719,
-8.65018508305617));
#73885=CARTESIAN_POINT('Ctrl Pts',(-19.4056288482904,-16.9443604719225,
-8.64996886196975));
#73886=CARTESIAN_POINT('Ctrl Pts',(-19.412890511726,-16.9468034089712,-8.64950443495672));
#73887=CARTESIAN_POINT('Ctrl Pts',(-19.4167594398678,-16.9481174579821,
-8.64925608244532));
#73888=CARTESIAN_POINT('Ctrl Pts',(-19.4273710689916,-16.9517559079326,
-8.64857244880002));
#73889=CARTESIAN_POINT('Ctrl Pts',(-19.4341057934348,-16.9541031703748,
-8.64813584824327));
#73890=CARTESIAN_POINT('Ctrl Pts',(-19.4695225241903,-16.9666480743012,
-8.64582592458136));
#73891=CARTESIAN_POINT('Ctrl Pts',(-19.4979923901222,-16.9774288928147,
-8.64392089889335));
#73892=CARTESIAN_POINT('Ctrl Pts',(-19.6765790273641,-17.0494953909534,
-8.63170746959015));
#73893=CARTESIAN_POINT('Ctrl Pts',(-19.8194665893621,-17.1272423355203,
-8.62079147907306));
#73894=CARTESIAN_POINT('Ctrl Pts',(-20.0499070855908,-17.289356180983,-8.60236922010302));
#73895=CARTESIAN_POINT('Ctrl Pts',(-20.1417396026641,-17.3663539203935,
-8.59474160483249));
#73896=CARTESIAN_POINT('Ctrl Pts',(-20.2377288060895,-17.461786767082,-8.58647641459699));
#73897=CARTESIAN_POINT('Ctrl Pts',(-20.2487462312271,-17.472986924435,-8.58552260796206));
#73898=CARTESIAN_POINT('Ctrl Pts',(-20.2652268079633,-17.4901181844641,
-8.58408768011977));
#73899=CARTESIAN_POINT('Ctrl Pts',(-20.2707822500935,-17.4959593760397,
-8.58360254227211));
#73900=CARTESIAN_POINT('Ctrl Pts',(-20.2806777377058,-17.506483573896,-8.58273575284525));
#73901=CARTESIAN_POINT('Ctrl Pts',(-20.2850301942227,-17.5111547270978,
-8.58235356858448));
#73902=CARTESIAN_POINT('Ctrl Pts',(-20.2942209522223,-17.5211083577414,
-8.58154450948689));
#73903=CARTESIAN_POINT('Ctrl Pts',(-20.2990537171269,-17.5263958557571,
-8.58111787344361));
#73904=CARTESIAN_POINT('Ctrl Pts',(-20.3088371014887,-17.5372095039485,
-8.58025166298613));
#73905=CARTESIAN_POINT('Ctrl Pts',(-20.3137856966663,-17.5427373563898,
-8.57981217681295));
#73906=CARTESIAN_POINT('Ctrl Pts',(-20.3355743469661,-17.567335468225,-8.57787098251012));
#73907=CARTESIAN_POINT('Ctrl Pts',(-20.3520993491615,-17.5866828819851,
-8.57638238057284));
#73908=CARTESIAN_POINT('Ctrl Pts',(-20.4222713890859,-17.6719041523003,
-8.56998126027263));
#73909=CARTESIAN_POINT('Ctrl Pts',(-20.4722775168634,-17.7406787622017,
-8.5652140362318));
#73910=CARTESIAN_POINT('Ctrl Pts',(-20.555189851896,-17.8704624298392,-8.55672638969621));
#73911=CARTESIAN_POINT('Ctrl Pts',(-20.5894925682938,-17.9304307782471,
-8.5529812588757));
#73912=CARTESIAN_POINT('Ctrl Pts',(-20.6801422890736,-18.1085898558519,
-8.54212539585322));
#73913=CARTESIAN_POINT('Ctrl Pts',(-20.728532700323,-18.2304457785093,-8.53503486061591));
#73914=CARTESIAN_POINT('Ctrl Pts',(-20.7697993273687,-18.3710882887299,
-8.52644202941237));
#73915=CARTESIAN_POINT('Ctrl Pts',(-20.7740668394217,-18.3862575008341,
-8.52550993438047));
#73916=CARTESIAN_POINT('Ctrl Pts',(-20.7796729212571,-18.4070734489269,
-8.52422185934865));
#73917=CARTESIAN_POINT('Ctrl Pts',(-20.781158322265,-18.4126805690425,-8.52387400541102));
#73918=CARTESIAN_POINT('Ctrl Pts',(-20.7834811070905,-18.4215965298827,
-8.52331936339071));
#73919=CARTESIAN_POINT('Ctrl Pts',(-20.7843335775881,-18.4249014611416,
-8.52311344120053));
#73920=CARTESIAN_POINT('Ctrl Pts',(-20.7860768719575,-18.4317282358,-8.52268737389335));
#73921=CARTESIAN_POINT('Ctrl Pts',(-20.7869666213985,-18.4352503046051,
-8.52246716590368));
#73922=CARTESIAN_POINT('Ctrl Pts',(-20.789063834877,-18.4436430230038,-8.52194152615588));
#73923=CARTESIAN_POINT('Ctrl Pts',(-20.7902630508741,-18.4485156944848,
-8.52163562321655));
#73924=CARTESIAN_POINT('Ctrl Pts',(-20.7927674030141,-18.4588496081269,
-8.52098539973067));
#73925=CARTESIAN_POINT('Ctrl Pts',(-20.7940681557944,-18.4643118613354,
-8.52064084111419));
#73926=CARTESIAN_POINT('Ctrl Pts',(-20.7975804743657,-18.4793259527679,
-8.51969149861464));
#73927=CARTESIAN_POINT('Ctrl Pts',(-20.799747407623,-18.4888879520619,-8.51908439180955));
#73928=CARTESIAN_POINT('Ctrl Pts',(-20.8343835371362,-18.6468077555266,
-8.50902050963056));
#73929=CARTESIAN_POINT('Ctrl Pts',(-20.850858530288,-18.7982035834032,-8.4988643478769));
#73930=CARTESIAN_POINT('Ctrl Pts',(-20.8509990928545,-18.950040190495,-8.48885786576293));
#73931=CARTESIAN_POINT('Ctrl Pts',(-20.8509991049198,-18.9500532671891,
-8.48905627902251));
#73932=CARTESIAN_POINT('Ctrl Pts',(-20.8510652694519,-19.0220047205605,
-8.48473008583432));
#73933=CARTESIAN_POINT('Ctrl Pts',(-20.8474590099796,-19.0940510985681,
-8.48040389264612));
#73934=CARTESIAN_POINT('Ctrl Pts',(-20.8401779985048,-19.1657831579297,
-8.47607769945793));
#73935=CARTESIAN_POINT('Ctrl Pts',(-20.8329019842481,-19.2374659850183,
-8.47175447549056));
#73936=CARTESIAN_POINT('Ctrl Pts',(-20.8219562717605,-19.3088344307463,
-8.46743125152319));
#73937=CARTESIAN_POINT('Ctrl Pts',(-20.8073905458149,-19.3794817475932,
-8.46310802755582));
#73938=CARTESIAN_POINT('Ctrl Pts',(-20.7928276075145,-19.4501155436823,
-8.45878563098384));
#73939=CARTESIAN_POINT('Ctrl Pts',(-20.774646124242,-19.5200279993613,-8.45446323441186));
#73940=CARTESIAN_POINT('Ctrl Pts',(-20.7529470567775,-19.5888216248916,
-8.45014083783989));
#73941=CARTESIAN_POINT('Ctrl Pts',(-20.7434887927382,-19.6188076266194,
-8.44825677677934));
#73942=CARTESIAN_POINT('Ctrl Pts',(-20.733362857865,-19.6485812163244,-8.4463727157188));
#73943=CARTESIAN_POINT('Ctrl Pts',(-20.7225805821191,-19.6781103693095,
-8.44448865465826));
#73944=CARTESIAN_POINT('Origin',(-18.734,-18.952,0.));
#73945=CARTESIAN_POINT('',(-20.7249098202513,-19.6789408942641,-7.64456002557215));
#73946=CARTESIAN_POINT('',(-20.7225805730004,-19.6781103942827,-7.86510594064262));
#73947=CARTESIAN_POINT('',(-20.7225805821191,-19.6781103693095,0.));
#73948=CARTESIAN_POINT('Ctrl Pts',(-20.7225805730004,-19.6781103942827,
-7.86510594064261));
#73949=CARTESIAN_POINT('Ctrl Pts',(-20.7375769517348,-19.6370401828501,
-7.86752231323783));
#73950=CARTESIAN_POINT('Ctrl Pts',(-20.7513004020704,-19.5955070040366,
-7.86996747030577));
#73951=CARTESIAN_POINT('Ctrl Pts',(-20.774507262156,-19.5172058397638,-7.87462975166453));
#73952=CARTESIAN_POINT('Ctrl Pts',(-20.7843049850557,-19.4805608708391,
-7.87683270548543));
#73953=CARTESIAN_POINT('Ctrl Pts',(-20.7948724739946,-19.4363047255142,
-7.8795398168314));
#73954=CARTESIAN_POINT('Ctrl Pts',(-20.7965927808939,-19.4289249809921,
-7.87999277135078));
#73955=CARTESIAN_POINT('Ctrl Pts',(-20.799201287806,-19.4174569185875,-7.88069927329126));
#73956=CARTESIAN_POINT('Ctrl Pts',(-20.8001170706691,-19.4133748495651,
-7.88095126622773));
#73957=CARTESIAN_POINT('Ctrl Pts',(-20.801790523728,-19.405810588006,-7.88141921480146));
#73958=CARTESIAN_POINT('Ctrl Pts',(-20.8025515035319,-19.4023291867746,
-7.88163497809511));
#73959=CARTESIAN_POINT('Ctrl Pts',(-20.8042489771272,-19.3944683368746,
-7.88212304445236));
#73960=CARTESIAN_POINT('Ctrl Pts',(-20.8051803610547,-19.3900878537022,
-7.88239563399139));
#73961=CARTESIAN_POINT('Ctrl Pts',(-20.8078797660236,-19.3771909821251,
-7.88319991817301));
#73962=CARTESIAN_POINT('Ctrl Pts',(-20.8096091831936,-19.3686667348037,
-7.88373373668598));
#73963=CARTESIAN_POINT('Ctrl Pts',(-20.8214936637338,-19.3081778481938,
-7.88753632508516));
#73964=CARTESIAN_POINT('Ctrl Pts',(-20.8297477276156,-19.255863294928,-7.89090073532048));
#73965=CARTESIAN_POINT('Ctrl Pts',(-20.8378088430684,-19.1884349094632,
-7.89528843836827));
#73966=CARTESIAN_POINT('Ctrl Pts',(-20.8394281650497,-19.1735521182162,
-7.89626010311883));
#73967=CARTESIAN_POINT('Ctrl Pts',(-20.8475637431883,-19.090607720525,-7.90168919291301));
#73968=CARTESIAN_POINT('Ctrl Pts',(-20.8509374103621,-19.0222802059237,
-7.90621179080917));
#73969=CARTESIAN_POINT('Ctrl Pts',(-20.8511442882594,-18.7931414079384,
-7.92135272976385));
#73970=CARTESIAN_POINT('Ctrl Pts',(-20.8329752262217,-18.6328491654654,
-7.9318507301475));
#73971=CARTESIAN_POINT('Ctrl Pts',(-20.7914795954939,-18.4529688454933,
-7.94322223271909));
#73972=CARTESIAN_POINT('Ctrl Pts',(-20.7857446846322,-18.4298906240303,
-7.94467451223104));
#73973=CARTESIAN_POINT('Ctrl Pts',(-20.7771304021409,-18.3975626272888,
-7.94670021104836));
#73974=CARTESIAN_POINT('Ctrl Pts',(-20.7745746984409,-18.3882291730159,
-7.94728403381575));
#73975=CARTESIAN_POINT('Ctrl Pts',(-20.7703333350992,-18.3731464462916,
-7.9482259155125));
#73976=CARTESIAN_POINT('Ctrl Pts',(-20.7686871312369,-18.3673863092582,
-7.94858525133491));
#73977=CARTESIAN_POINT('Ctrl Pts',(-20.7652024825499,-18.3553863998426,
-7.94933309843104));
#73978=CARTESIAN_POINT('Ctrl Pts',(-20.7633596821685,-18.3491479494473,
-7.94972146322238));
#73979=CARTESIAN_POINT('Ctrl Pts',(-20.7589304691935,-18.3344041590598,
-7.9506383625105));
#73980=CARTESIAN_POINT('Ctrl Pts',(-20.7563191658415,-18.3259063784405,
-7.95116607717529));
#73981=CARTESIAN_POINT('Ctrl Pts',(-20.7474528216397,-18.2976875603047,
-7.9529161589399));
#73982=CARTESIAN_POINT('Ctrl Pts',(-20.7409621037977,-18.2780414015876,
-7.95413078979751));
#73983=CARTESIAN_POINT('Ctrl Pts',(-20.7048338630199,-18.173841818229,-7.96055734970913));
#73984=CARTESIAN_POINT('Ctrl Pts',(-20.6701375509487,-18.0911339775254,
-7.96559785907302));
#73985=CARTESIAN_POINT('Ctrl Pts',(-20.5703572778889,-17.8900856685431,
-7.97797948641753));
#73986=CARTESIAN_POINT('Ctrl Pts',(-20.4990150235356,-17.7753139913978,
-7.98515792929512));
#73987=CARTESIAN_POINT('Ctrl Pts',(-20.3708542712837,-17.6072887135831,
-7.99685019316134));
#73988=CARTESIAN_POINT('Ctrl Pts',(-20.3212057823279,-17.5490333233624,
-8.00116977687783));
#73989=CARTESIAN_POINT('Ctrl Pts',(-20.2619779474793,-17.4867141577325,
-8.00626515299267));
#73990=CARTESIAN_POINT('Ctrl Pts',(-20.2553888188801,-17.4798738974814,
-8.00683128284337));
#73991=CARTESIAN_POINT('Ctrl Pts',(-20.2455537549553,-17.4698005425575,
-8.00767564233198));
#73992=CARTESIAN_POINT('Ctrl Pts',(-20.2423428880607,-17.4665331653336,
-8.00795119911209));
#73993=CARTESIAN_POINT('Ctrl Pts',(-20.2366096484543,-17.4607367761918,
-8.00844310129746));
#73994=CARTESIAN_POINT('Ctrl Pts',(-20.2340914555426,-17.458203700939,-8.00865911766408));
#73995=CARTESIAN_POINT('Ctrl Pts',(-20.2286618090162,-17.4527695410695,
-8.00912481463519));
#73996=CARTESIAN_POINT('Ctrl Pts',(-20.2257483568813,-17.4498706009819,
-8.00937465080113));
#73997=CARTESIAN_POINT('Ctrl Pts',(-20.2176786552267,-17.441887725482,-8.0100664663301));
#73998=CARTESIAN_POINT('Ctrl Pts',(-20.2125047915287,-17.4368217888439,
-8.01050981701182));
#73999=CARTESIAN_POINT('Ctrl Pts',(-20.1839451825361,-17.4091434990124,
-8.01295545762008));
#74000=CARTESIAN_POINT('Ctrl Pts',(-20.1600679703785,-17.3870472563484,
-8.01499407407326));
#74001=CARTESIAN_POINT('Ctrl Pts',(-20.0137581027677,-17.2577797178948,
-8.02739994363735));
#74002=CARTESIAN_POINT('Ctrl Pts',(-19.8798138969812,-17.1644671727211,
-8.03835720679495));
#74003=CARTESIAN_POINT('Ctrl Pts',(-19.6336216902987,-17.0321003208917,
-8.05661529396626));
#74004=CARTESIAN_POINT('Ctrl Pts',(-19.5263234516695,-16.9853873493609,
-8.06405613720958));
#74005=CARTESIAN_POINT('Ctrl Pts',(-19.4021738928779,-16.9431603263832,
-8.072063197309));
#74006=CARTESIAN_POINT('Ctrl Pts',(-19.3885991738552,-16.9386959686313,
-8.07293117340852));
#74007=CARTESIAN_POINT('Ctrl Pts',(-19.3669223584555,-16.93180947261,-8.0743054820485));
#74008=CARTESIAN_POINT('Ctrl Pts',(-19.3588493379269,-16.9292978996104,
-8.07481474265757));
#74009=CARTESIAN_POINT('Ctrl Pts',(-19.3445847677139,-16.9249536436865,
-8.07571012077674));
#74010=CARTESIAN_POINT('Ctrl Pts',(-19.3383995141151,-16.9231008112825,
-8.07609689441409));
#74011=CARTESIAN_POINT('Ctrl Pts',(-19.3255888935864,-16.9193270887387,
-8.07689496309716));
#74012=CARTESIAN_POINT('Ctrl Pts',(-19.3189624135805,-16.9174102232587,
-8.07730612276231));
#74013=CARTESIAN_POINT('Ctrl Pts',(-19.3019291090047,-16.9125730329247,
-8.07835883230764));
#74014=CARTESIAN_POINT('Ctrl Pts',(-19.2915089929618,-16.9096999348249,
-8.0789988408874));
#74015=CARTESIAN_POINT('Ctrl Pts',(-19.2479272925843,-16.8980417291663,
-8.08165950425955));
#74016=CARTESIAN_POINT('Ctrl Pts',(-19.2145755511478,-16.88998322591,-8.08365663035751));
#74017=CARTESIAN_POINT('Ctrl Pts',(-19.1271789034915,-16.8711021398066,
-8.08880070168368));
#74018=CARTESIAN_POINT('Ctrl Pts',(-19.0728803418643,-16.8615726958346,
-8.09190825804238));
#74019=CARTESIAN_POINT('Ctrl Pts',(-18.9099125905281,-16.8394895540177,
-8.10105266393844));
#74020=CARTESIAN_POINT('Ctrl Pts',(-18.8005788010384,-16.8332235203395,
-8.10694078407108));
#74021=CARTESIAN_POINT('Ctrl Pts',(-18.6455318676336,-16.836355073568,-8.11538391013854));
#74022=CARTESIAN_POINT('Ctrl Pts',(-18.5998561999474,-16.8387595335954,
-8.11788423302371));
#74023=CARTESIAN_POINT('Ctrl Pts',(-18.5315832706288,-16.8445759646648,
-8.12168371900076));
#74024=CARTESIAN_POINT('Ctrl Pts',(-18.5089041621511,-16.846877578628,-8.12295622388119));
#74025=CARTESIAN_POINT('Ctrl Pts',(-18.4852295120212,-16.8496671680906,
-8.12429937232324));
#74026=CARTESIAN_POINT('Ctrl Pts',(-18.4841918842235,-16.8497902109685,
-8.12435827048077));
#74027=CARTESIAN_POINT('Ctrl Pts',(-18.4647180185559,-16.8521140619218,
-8.12546421814634));
#74028=CARTESIAN_POINT('Ctrl Pts',(-18.4463119143648,-16.8545564925169,
-8.12651904434817));
#74029=CARTESIAN_POINT('Ctrl Pts',(-18.3950051768962,-16.8620527702356,
-8.12949177821453));
#74030=CARTESIAN_POINT('Ctrl Pts',(-18.3621896439015,-16.8676406991701,
-8.1314305004841));
#74031=CARTESIAN_POINT('Ctrl Pts',(-18.322734327069,-16.8753205932203,-8.1338215071503));
#74032=CARTESIAN_POINT('Ctrl Pts',(-18.3159536859165,-16.8766749438753,
-8.13423457153015));
#74033=CARTESIAN_POINT('Ctrl Pts',(-18.3048275232537,-16.8789539987548,
-8.13491608070141));
#74034=CARTESIAN_POINT('Ctrl Pts',(-18.3004780020547,-16.8798592194194,
-8.13518343811733));
#74035=CARTESIAN_POINT('Ctrl Pts',(-18.2926468243224,-16.8815147768423,
-8.13566654829429));
#74036=CARTESIAN_POINT('Ctrl Pts',(-18.2891641881197,-16.8822602131825,
-8.13588201867212));
#74037=CARTESIAN_POINT('Ctrl Pts',(-18.2815669855834,-16.8839064073329,
-8.13635343036611));
#74038=CARTESIAN_POINT('Ctrl Pts',(-18.2774532718618,-16.8848106460998,
-8.13660956455088));
#74039=CARTESIAN_POINT('Ctrl Pts',(-18.2658181950799,-16.8874045859091,
-8.13733643035061));
#74040=CARTESIAN_POINT('Ctrl Pts',(-18.2583034150761,-16.8891230814121,
-8.13780876561804));
#74041=CARTESIAN_POINT('Ctrl Pts',(-18.2115398945837,-16.900086169211,-8.14076524566598));
#74042=CARTESIAN_POINT('Ctrl Pts',(-18.1725552912503,-16.9104088851109,
-8.14330544084794));
#74043=CARTESIAN_POINT('Ctrl Pts',(-17.9653010190008,-16.971672398734,-8.1571325318623));
#74044=CARTESIAN_POINT('Ctrl Pts',(-17.8035730229403,-17.0423123962943,
-8.16900644133708));
#74045=CARTESIAN_POINT('Ctrl Pts',(-17.5700156459866,-17.1811185658956,
-8.18659640531032));
#74046=CARTESIAN_POINT('Ctrl Pts',(-17.4910131495683,-17.2356466705537,
-8.19265270697207));
#74047=CARTESIAN_POINT('Ctrl Pts',(-17.4051166463315,-17.3039859247083,
-8.19935130705287));
#74048=CARTESIAN_POINT('Ctrl Pts',(-17.3943481380458,-17.3127275201632,
-8.2001934366143));
#74049=CARTESIAN_POINT('Ctrl Pts',(-17.3772490422362,-17.3268891535833,
-8.20153464069264));
#74050=CARTESIAN_POINT('Ctrl Pts',(-17.370863337019,-17.3322417261605,-8.20203642783339));
#74051=CARTESIAN_POINT('Ctrl Pts',(-17.3596004320728,-17.3417962035236,
-8.20292314923341));
#74052=CARTESIAN_POINT('Ctrl Pts',(-17.3547105149916,-17.3459828903557,
-8.20330869966901));
#74053=CARTESIAN_POINT('Ctrl Pts',(-17.3445808641742,-17.354736160995,-8.2041086115322));
#74054=CARTESIAN_POINT('Ctrl Pts',(-17.3393443636244,-17.3593063809733,
-8.20452281594534));
#74055=CARTESIAN_POINT('Ctrl Pts',(-17.325844191368,-17.3712064555667,-8.20559253814179));
#74056=CARTESIAN_POINT('Ctrl Pts',(-17.3176151432258,-17.3785754050474,
-8.20624641573205));
#74057=CARTESIAN_POINT('Ctrl Pts',(-17.2824963105024,-17.410522413642,-8.20904535830756));
#74058=CARTESIAN_POINT('Ctrl Pts',(-17.256184752552,-17.4357287715275,-8.2111636585819));
#74059=CARTESIAN_POINT('Ctrl Pts',(-17.1883711243933,-17.5041369617202,
-8.21669533302375));
#74060=CARTESIAN_POINT('Ctrl Pts',(-17.1480286396272,-17.5484432187357,
-8.22006106370756));
#74061=CARTESIAN_POINT('Ctrl Pts',(-17.0021949425094,-17.7229352452395,
-8.23265905147324));
#74062=CARTESIAN_POINT('Ctrl Pts',(-16.9104175366594,-17.8637498711217,
-8.2414764740787));
#74063=CARTESIAN_POINT('Ctrl Pts',(-16.8122471860583,-18.0623502935211,
-8.25392823211294));
#74064=CARTESIAN_POINT('Ctrl Pts',(-16.7901623422886,-18.1116997069089,
-8.25702817247595));
#74065=CARTESIAN_POINT('Ctrl Pts',(-16.7667270226798,-18.1699497858908,
-8.26075397809295));
#74066=CARTESIAN_POINT('Ctrl Pts',(-16.7635127260228,-18.1780843703571,
-8.26127576974325));
#74067=CARTESIAN_POINT('Ctrl Pts',(-16.7587252588649,-18.1904234460761,
-8.26206983659402));
#74068=CARTESIAN_POINT('Ctrl Pts',(-16.7571148562181,-18.1946135214474,
-8.26233993182966));
#74069=CARTESIAN_POINT('Ctrl Pts',(-16.7542496742715,-18.2021397780864,
-8.26282593603129));
#74070=CARTESIAN_POINT('Ctrl Pts',(-16.7529899839128,-18.2054740322665,
-8.26304154698378));
#74071=CARTESIAN_POINT('Ctrl Pts',(-16.7502728584379,-18.2127212550191,
-8.2635108614417));
#74072=CARTESIAN_POINT('Ctrl Pts',(-16.7488185970028,-18.2166353071776,
-8.26376474461393));
#74073=CARTESIAN_POINT('Ctrl Pts',(-16.7447705687403,-18.2276298384392,
-8.26447901828793));
#74074=CARTESIAN_POINT('Ctrl Pts',(-16.7422030695044,-18.2347198281789,
-8.26494092708758));
#74075=CARTESIAN_POINT('Ctrl Pts',(-16.7271661854344,-18.2769465781668,
-8.26769903644834));
#74076=CARTESIAN_POINT('Ctrl Pts',(-16.7155897347785,-18.3123917691351,
-8.27004310493703));
#74077=CARTESIAN_POINT('Ctrl Pts',(-16.680740099376,-18.4294872443724,-8.27783956209834));
#74078=CARTESIAN_POINT('Ctrl Pts',(-16.6614419056787,-18.5122308727529,
-8.28342858341367));
#74079=CARTESIAN_POINT('Ctrl Pts',(-16.6171404602724,-18.7718509713058,
-8.30082694090861));
#74080=CARTESIAN_POINT('Ctrl Pts',(-16.6094832357551,-18.9509273227642,
-8.31255834900709));
#74081=CARTESIAN_POINT('Ctrl Pts',(-16.6263017938675,-19.1515369502787,
-8.32494667262787));
#74082=CARTESIAN_POINT('Ctrl Pts',(-16.628568198236,-19.1741794639391,-8.32633548483591));
#74083=CARTESIAN_POINT('Ctrl Pts',(-16.6322985450934,-19.2062250553771,
-8.32828832310606));
#74084=CARTESIAN_POINT('Ctrl Pts',(-16.6334614295865,-19.2156609625164,
-8.32886177544001));
#74085=CARTESIAN_POINT('Ctrl Pts',(-16.6354566483555,-19.2309987808936,
-8.32979143955576));
#74086=CARTESIAN_POINT('Ctrl Pts',(-16.6362504017109,-19.2369054974522,
-8.330148864309));
#74087=CARTESIAN_POINT('Ctrl Pts',(-16.6379662154926,-19.249277690343,-8.33089630464623));
#74088=CARTESIAN_POINT('Ctrl Pts',(-16.6388932735334,-19.2557424190993,
-8.33128615804059));
#74089=CARTESIAN_POINT('Ctrl Pts',(-16.641173991873,-19.2711393323343,-8.33221304448785));
#74090=CARTESIAN_POINT('Ctrl Pts',(-16.6425549484176,-19.2800673921619,
-8.33274920782139));
#74091=CARTESIAN_POINT('Ctrl Pts',(-16.647421065704,-19.3102472975736,-8.33455742314247));
#74092=CARTESIAN_POINT('Ctrl Pts',(-16.6511734077091,-19.3314551515858,
-8.33582100452812));
#74093=CARTESIAN_POINT('Ctrl Pts',(-16.6894830919419,-19.5302464016374,
-8.34760783215506));
#74094=CARTESIAN_POINT('Ctrl Pts',(-16.7463443575211,-19.7027663999737,
-8.35731961999596));
#74095=CARTESIAN_POINT('Ctrl Pts',(-16.8344242330958,-19.8867908148481,
-8.368426120785));
#74096=CARTESIAN_POINT('Ctrl Pts',(-16.844730935649,-19.9074498114198,-8.36968569531807));
#74097=CARTESIAN_POINT('Ctrl Pts',(-16.8994260274842,-20.0127350664337,
-8.37618922527099));
#74098=CARTESIAN_POINT('Ctrl Pts',(-16.9491644025574,-20.0944437469731,
-8.3815173085108));
#74099=CARTESIAN_POINT('Ctrl Pts',(-17.0098276787814,-20.1804187650058,
-8.38775119259468));
#74100=CARTESIAN_POINT('Ctrl Pts',(-17.0154671465867,-20.1882959512832,
-8.38832850850654));
#74101=CARTESIAN_POINT('Ctrl Pts',(-17.0238743864598,-20.1998704713225,
-8.38918638145135));
#74102=CARTESIAN_POINT('Ctrl Pts',(-17.0266006026634,-20.2035980282553,
-8.3894641399494));
#74103=CARTESIAN_POINT('Ctrl Pts',(-17.0314591743147,-20.2101957405938,
-8.38995846111537));
#74104=CARTESIAN_POINT('Ctrl Pts',(-17.0335866272514,-20.2130694454873,
-8.39017468227016));
#74105=CARTESIAN_POINT('Ctrl Pts',(-17.0381609035332,-20.2192156305914,
-8.39063910886491));
#74106=CARTESIAN_POINT('Ctrl Pts',(-17.0406098869413,-20.2224863713803,
-8.39088746088674));
#74107=CARTESIAN_POINT('Ctrl Pts',(-17.0473595113515,-20.2314466494183,
-8.39157109184889));
#74108=CARTESIAN_POINT('Ctrl Pts',(-17.0516794132692,-20.2371215144025,
-8.39200769019514));
#74109=CARTESIAN_POINT('Ctrl Pts',(-17.0749154365423,-20.2673277237891,
-8.39435060087743));
#74110=CARTESIAN_POINT('Ctrl Pts',(-17.0943385641695,-20.2914621126119,
-8.3962898044529));
#74111=CARTESIAN_POINT('Ctrl Pts',(-17.2195873812324,-20.4402836910671,
-8.40863151368927));
#74112=CARTESIAN_POINT('Ctrl Pts',(-17.3390319459713,-20.5527803351579,
-8.41964613513472));
#74113=CARTESIAN_POINT('Ctrl Pts',(-17.5646709594519,-20.7206760457512,
-8.4380232878025));
#74114=CARTESIAN_POINT('Ctrl Pts',(-17.6648165734466,-20.7829560725207,
-8.44552423348077));
#74115=CARTESIAN_POINT('Ctrl Pts',(-17.782369035971,-20.843108684175,-8.45358726558593));
#74116=CARTESIAN_POINT('Ctrl Pts',(-17.7951668753124,-20.8494946447379,
-8.45445602036142));
#74117=CARTESIAN_POINT('Ctrl Pts',(-17.8156348684865,-20.859450137226,-8.45583132493096));
#74118=CARTESIAN_POINT('Ctrl Pts',(-17.8232632265163,-20.8631041503412,
-8.45634080939984));
#74119=CARTESIAN_POINT('Ctrl Pts',(-17.8367536640226,-20.8694670035107,
-8.45723644793592));
#74120=CARTESIAN_POINT('Ctrl Pts',(-17.8426065837236,-20.8721949056878,
-8.45762325933131));
#74121=CARTESIAN_POINT('Ctrl Pts',(-17.8547361793791,-20.8777808017584,
-8.45842127846437));
#74122=CARTESIAN_POINT('Ctrl Pts',(-17.8610145302108,-20.8806349924083,
-8.45883235144981));
#74123=CARTESIAN_POINT('Ctrl Pts',(-17.8771619324139,-20.8878807314515,
-8.45988457537688));
#74124=CARTESIAN_POINT('Ctrl Pts',(-17.8870509275065,-20.8922275525357,
-8.46052418780893));
#74125=CARTESIAN_POINT('Ctrl Pts',(-17.9284285662296,-20.9100389336873,
-8.46318100360758));
#74126=CARTESIAN_POINT('Ctrl Pts',(-17.9602093615057,-20.9228145636113,
-8.46517476504808));
#74127=CARTESIAN_POINT('Ctrl Pts',(-18.0437776850987,-20.9540750178992,
-8.47030821499117));
#74128=CARTESIAN_POINT('Ctrl Pts',(-18.0960008937031,-20.9713238975377,
-8.47340872758479));
#74129=CARTESIAN_POINT('Ctrl Pts',(-18.2538216920665,-21.0167156670898,
-8.4825408426409));
#74130=CARTESIAN_POINT('Ctrl Pts',(-18.3609865215301,-21.0387400016039,
-8.48842367542667));
#74131=CARTESIAN_POINT('Ctrl Pts',(-18.5016775786826,-21.0564656108686,
-8.4961435522461));
#74132=CARTESIAN_POINT('Ctrl Pts',(-18.5340722027113,-21.0597898422532,
-8.49792169480362));
#74133=CARTESIAN_POINT('Ctrl Pts',(-18.6522825775706,-21.0691705350073,
-8.50444936866397));
#74134=CARTESIAN_POINT('Ctrl Pts',(-18.7383602080486,-21.0707416539178,
-8.50927612889432));
#74135=CARTESIAN_POINT('Ctrl Pts',(-18.8338936818678,-21.0666637516451,
-8.51494188325393));
#74136=CARTESIAN_POINT('Ctrl Pts',(-18.8435010798833,-21.0661880322748,
-8.51551516134385));
#74137=CARTESIAN_POINT('Ctrl Pts',(-18.8577021944282,-21.0653877947978,
-8.5163681587277));
#74138=CARTESIAN_POINT('Ctrl Pts',(-18.8622987852553,-21.0651137273914,
-8.51664512516844));
#74139=CARTESIAN_POINT('Ctrl Pts',(-18.8704615536325,-21.0646002980545,
-8.51713857360574));
#74140=CARTESIAN_POINT('Ctrl Pts',(-18.8740280567105,-21.0643668994937,
-8.51735471857563));
#74141=CARTESIAN_POINT('Ctrl Pts',(-18.8816790799238,-21.063846740259,-8.517819590728));
#74142=CARTESIAN_POINT('Ctrl Pts',(-18.8857633031915,-21.0635571657281,
-8.51806846767783));
#74143=CARTESIAN_POINT('Ctrl Pts',(-18.8969977639433,-21.0627278712461,
-8.51875499058577));
#74144=CARTESIAN_POINT('Ctrl Pts',(-18.9041460619185,-21.0621636741561,
-8.51919397419287));
#74145=CARTESIAN_POINT('Ctrl Pts',(-18.9426968143835,-21.0589238041009,
-8.52157257020084));
#74146=CARTESIAN_POINT('Ctrl Pts',(-18.9740376418705,-21.055583599726,-8.52354624705379));
#74147=CARTESIAN_POINT('Ctrl Pts',(-19.1675181476385,-21.0305832503529,
-8.53593094290034));
#74148=CARTESIAN_POINT('Ctrl Pts',(-19.3267651978501,-20.9908907591632,
-8.54694858740966));
#74149=CARTESIAN_POINT('Ctrl Pts',(-19.5894103359619,-20.8920170109195,
-8.56528158817152));
#74150=CARTESIAN_POINT('Ctrl Pts',(-19.6953717245056,-20.8417526575434,
-8.57273930452554));
#74151=CARTESIAN_POINT('Ctrl Pts',(-19.8101120405206,-20.7751605038146,
-8.5808399341808));
#74152=CARTESIAN_POINT('Ctrl Pts',(-19.8234898862179,-20.7671978279436,
-8.58178512023024));
#74153=CARTESIAN_POINT('Ctrl Pts',(-19.8435544307931,-20.7549534015224,
-8.58320410595264));
#74154=CARTESIAN_POINT('Ctrl Pts',(-19.8503066561389,-20.7507805466739,
-8.58368186786966));
#74155=CARTESIAN_POINT('Ctrl Pts',(-19.8622901834543,-20.7432812982607,
-8.58453025648648));
#74156=CARTESIAN_POINT('Ctrl Pts',(-19.8675306149866,-20.7399697351279,
-8.5849014242043));
#74157=CARTESIAN_POINT('Ctrl Pts',(-19.8777828624621,-20.7334278865183,
-8.58562792440446));
#74158=CARTESIAN_POINT('Ctrl Pts',(-19.8827957227794,-20.7301993532136,
-8.58598331723653));
#74159=CARTESIAN_POINT('Ctrl Pts',(-19.8965063352287,-20.7212868554088,
-8.5869558567801));
#74160=CARTESIAN_POINT('Ctrl Pts',(-19.9051760618663,-20.7155599207609,
-8.58757139381875));
#74161=CARTESIAN_POINT('Ctrl Pts',(-19.9394052752561,-20.6925854941156,
-8.59000424639734));
#74162=CARTESIAN_POINT('Ctrl Pts',(-19.9646295784435,-20.6748437900011,
-8.591802869364));
#74163=CARTESIAN_POINT('Ctrl Pts',(-20.0278333115618,-20.6282923009128,
-8.59633269942516));
#74164=CARTESIAN_POINT('Ctrl Pts',(-20.0652445440261,-20.5987388751438,
-8.59903571713064));
#74165=CARTESIAN_POINT('Ctrl Pts',(-20.2548236585266,-20.4382918613778,
-8.61293427422033));
#74166=CARTESIAN_POINT('Ctrl Pts',(-20.3887826666009,-20.2875321456035,
-8.6233575791137));
#74167=CARTESIAN_POINT('Ctrl Pts',(-20.5222696864977,-20.0857910118521,
-8.63711213022692));
#74168=CARTESIAN_POINT('Ctrl Pts',(-20.5440198585186,-20.0507347895498,
-8.6395001000153));
#74169=CARTESIAN_POINT('Ctrl Pts',(-20.5684453767921,-20.0086711334096,
-8.6423902045905));
#74170=CARTESIAN_POINT('Ctrl Pts',(-20.5721265261176,-20.0022545381827,
-8.6428317414232));
#74171=CARTESIAN_POINT('Ctrl Pts',(-20.578037029276,-19.9918257074463,-8.64355066140592));
#74172=CARTESIAN_POINT('Ctrl Pts',(-20.5802871333345,-19.9878252205756,
-8.64382674485742));
#74173=CARTESIAN_POINT('Ctrl Pts',(-20.5842655206248,-19.9806978504854,
-8.64431922367947));
#74174=CARTESIAN_POINT('Ctrl Pts',(-20.5859989159615,-19.9775738781084,
-8.64453528702635));
#74175=CARTESIAN_POINT('Ctrl Pts',(-20.5897066045093,-19.97085172727,-8.64500067096878));
#74176=CARTESIAN_POINT('Ctrl Pts',(-20.5916783155431,-19.9672522442628,
-8.64525014494193));
#74177=CARTESIAN_POINT('Ctrl Pts',(-20.5970870909802,-19.957309673638,-8.64593996075882));
#74178=CARTESIAN_POINT('Ctrl Pts',(-20.600502179122,-19.9509547839456,-8.64638166115672));
#74179=CARTESIAN_POINT('Ctrl Pts',(-20.6189552149497,-19.9161918873852,
-8.64880170059864));
#74180=CARTESIAN_POINT('Ctrl Pts',(-20.6333762963376,-19.8874632985264,
-8.65081549346985));
#74181=CARTESIAN_POINT('Ctrl Pts',(-20.6750700256576,-19.7994623073921,
-8.6570009759816));
#74182=CARTESIAN_POINT('Ctrl Pts',(-20.7002399655389,-19.7392940263136,
-8.66125187701144));
#74183=CARTESIAN_POINT('Ctrl Pts',(-20.7225804318258,-19.6781107809139,
-8.66553671816755));
#74184=CARTESIAN_POINT('',(-20.8507519460844,-18.9524633045424,-7.68905625084234));
#74185=CARTESIAN_POINT('Ctrl Pts',(-20.7225805821191,-19.6781103693095,
-8.44448865465826));
#74186=CARTESIAN_POINT('Ctrl Pts',(-20.697822657537,-19.7459142874996,-8.44016253253484));
#74187=CARTESIAN_POINT('Ctrl Pts',(-20.6696010727523,-19.8124278882354,
-8.43583641041142));
#74188=CARTESIAN_POINT('Ctrl Pts',(-20.6380875232199,-19.8772781765061,
-8.431510288288));
#74189=CARTESIAN_POINT('Ctrl Pts',(-20.6065602995994,-19.9421566040554,
-8.42718228901091));
#74190=CARTESIAN_POINT('Ctrl Pts',(-20.5717385063017,-20.0053698483387,
-8.42285428973383));
#74191=CARTESIAN_POINT('Ctrl Pts',(-20.5338393726596,-20.0665704251524,
-8.41852629045674));
#74192=CARTESIAN_POINT('Ctrl Pts',(-20.4958706164931,-20.1278834303579,
-8.41419034043762));
#74193=CARTESIAN_POINT('Ctrl Pts',(-20.454813509682,-20.1871759749339,-8.4098543904185));
#74194=CARTESIAN_POINT('Ctrl Pts',(-20.4109277577034,-20.244130912657,-8.40551844039938));
#74195=CARTESIAN_POINT('Ctrl Pts',(-20.3707283792957,-20.2963016740203,
-8.40154670725781));
#74196=CARTESIAN_POINT('Ctrl Pts',(-20.3281562877958,-20.3465112289193,
-8.39757497411623));
#74197=CARTESIAN_POINT('Ctrl Pts',(-20.2834377820476,-20.3945434342034,
-8.39360324097466));
#74198=CARTESIAN_POINT('Ctrl Pts',(-20.234030095452,-20.447612294745,-8.38921503204376));
#74199=CARTESIAN_POINT('Ctrl Pts',(-20.1817963672774,-20.4982434590661,
-8.38482682311287));
#74200=CARTESIAN_POINT('Ctrl Pts',(-20.1270066890246,-20.5461208750697,
-8.38043861418197));
#74201=CARTESIAN_POINT('Ctrl Pts',(-20.0722983277385,-20.5939272330497,
-8.3760569180807));
#74202=CARTESIAN_POINT('Ctrl Pts',(-20.01504190713,-20.6389876412174,-8.37167522197942));
#74203=CARTESIAN_POINT('Ctrl Pts',(-19.9555455237306,-20.6810215537852,
-8.36729352587815));
#74204=CARTESIAN_POINT('Ctrl Pts',(-19.8961190533168,-20.7230060731604,
-8.36291697861851));
#74205=CARTESIAN_POINT('Ctrl Pts',(-19.8344582408823,-20.7619708847354,
-8.35854043135888));
#74206=CARTESIAN_POINT('Ctrl Pts',(-19.7709042257784,-20.7976756558407,
-8.35416388409924));
#74207=CARTESIAN_POINT('Ctrl Pts',(-19.7073905157073,-20.833357783499,-8.34979011238226));
#74208=CARTESIAN_POINT('Ctrl Pts',(-19.6419864047148,-20.8657837371301,
-8.34541634066529));
#74209=CARTESIAN_POINT('Ctrl Pts',(-19.5750607832523,-20.8947572568067,
-8.34104256894831));
#74210=CARTESIAN_POINT('Ctrl Pts',(-19.5081555274813,-20.9237219597439,
-8.33667012818477));
#74211=CARTESIAN_POINT('Ctrl Pts',(-19.4397301228484,-20.9492361229378,
-8.33229768742123));
#74212=CARTESIAN_POINT('Ctrl Pts',(-19.3701752330597,-20.9711508296414,
-8.32792524665768));
#74213=CARTESIAN_POINT('Ctrl Pts',(-19.3006185647447,-20.9930660967064,
-8.32355269409035));
#74214=CARTESIAN_POINT('Ctrl Pts',(-19.2299328146161,-21.0113815814961,
-8.31918014152301));
#74215=CARTESIAN_POINT('Ctrl Pts',(-19.158524056411,-21.0259981498372,-8.31480758895567));
#74216=CARTESIAN_POINT('Ctrl Pts',(-19.0870411875032,-21.0406298878043,
-8.31043049838835));
#74217=CARTESIAN_POINT('Ctrl Pts',(-19.0148342859549,-21.0515549478116,
-8.30605340782102));
#74218=CARTESIAN_POINT('Ctrl Pts',(-18.9423190546122,-21.0587254618211,
-8.3016763172537));
#74219=CARTESIAN_POINT('Ctrl Pts',(-18.8697642200103,-21.0658998919145,
-8.29729683619476));
#74220=CARTESIAN_POINT('Ctrl Pts',(-18.7969012025329,-21.0693156708866,
-8.29291735513582));
#74221=CARTESIAN_POINT('Ctrl Pts',(-18.724147530365,-21.0689770732916,-8.28853787407688));
#74222=CARTESIAN_POINT('Ctrl Pts',(-18.6512649028016,-21.0686378755345,
-8.28415063041716));
#74223=CARTESIAN_POINT('Ctrl Pts',(-18.5784924896217,-21.0645310394331,
-8.27976338675744));
#74224=CARTESIAN_POINT('Ctrl Pts',(-18.506243930903,-21.0567128481077,-8.27537614309772));
#74225=CARTESIAN_POINT('Ctrl Pts',(-18.4571218728287,-21.0513972313654,
-8.2723932401629));
#74226=CARTESIAN_POINT('Ctrl Pts',(-18.408241843936,-21.0443670563134,-8.26941033722807));
#74227=CARTESIAN_POINT('Ctrl Pts',(-18.3597305432933,-21.0356533717911,
-8.26642743429324));
#74228=CARTESIAN_POINT('Ctrl Pts',(-18.2883645862438,-21.0228344939807,
-8.26203922536235));
#74229=CARTESIAN_POINT('Ctrl Pts',(-18.2175186632354,-21.0063198837036,
-8.25765101643146));
#74230=CARTESIAN_POINT('Ctrl Pts',(-18.147604719472,-20.9861655721633,-8.25326280750056));
#74231=CARTESIAN_POINT('Ctrl Pts',(-18.0777945395931,-20.966041172963,-8.2488811113993));
#74232=CARTESIAN_POINT('Ctrl Pts',(-18.008914052767,-20.9422879285592,-8.24449941529804));
#74233=CARTESIAN_POINT('Ctrl Pts',(-17.9413659204126,-20.915013045264,-8.24011771919678));
#74234=CARTESIAN_POINT('Ctrl Pts',(-17.8738971624894,-20.8877702121273,
-8.23574117193714));
#74235=CARTESIAN_POINT('Ctrl Pts',(-17.807758093989,-20.8570141403844,-8.2313646246775));
#74236=CARTESIAN_POINT('Ctrl Pts',(-17.7433354489135,-20.8229015867278,
-8.22698807741786));
#74237=CARTESIAN_POINT('Ctrl Pts',(-17.6789536597432,-20.7888106667569,
-8.22261430570089));
#74238=CARTESIAN_POINT('Ctrl Pts',(-17.6162865594647,-20.7513677135309,
-8.21824053398391));
#74239=CARTESIAN_POINT('Ctrl Pts',(-17.5556988450228,-20.7107766737648,
-8.21386676226694));
#74240=CARTESIAN_POINT('Ctrl Pts',(-17.4951295676258,-20.6701979859885,
-8.20949432150338));
#74241=CARTESIAN_POINT('Ctrl Pts',(-17.436638820346,-20.6264733818697,-8.20512188073983));
#74242=CARTESIAN_POINT('Ctrl Pts',(-17.3805632774559,-20.5798507419506,
-8.20074943997627));
#74243=CARTESIAN_POINT('Ctrl Pts',(-17.3244863007081,-20.5332269098855,
-8.19637688740893));
#74244=CARTESIAN_POINT('Ctrl Pts',(-17.2708250206049,-20.4837052048259,
-8.1920043348416));
#74245=CARTESIAN_POINT('Ctrl Pts',(-17.2198825933099,-20.4315734110743,
-8.18763178227426));
#74246=CARTESIAN_POINT('Ctrl Pts',(-17.1688872960423,-20.3793875129808,
-8.18325469170693));
#74247=CARTESIAN_POINT('Ctrl Pts',(-17.1206168232086,-20.3245864635404,
-8.17887760113961));
#74248=CARTESIAN_POINT('Ctrl Pts',(-17.0753364363194,-20.2674938929992,
-8.17450051057228));
#74249=CARTESIAN_POINT('Ctrl Pts',(-17.0300313201303,-20.2103701420863,
-8.17012102951334));
#74250=CARTESIAN_POINT('Ctrl Pts',(-16.9877198211694,-20.1509527715826,
-8.1657415484544));
#74251=CARTESIAN_POINT('Ctrl Pts',(-16.9486243453007,-20.0895951703514,
-8.16136206739546));
#74252=CARTESIAN_POINT('Ctrl Pts',(-16.9094595729634,-20.028128813184,-8.15697482373574));
#74253=CARTESIAN_POINT('Ctrl Pts',(-16.8735224451874,-19.9647157776944,
-8.15258758007602));
#74254=CARTESIAN_POINT('Ctrl Pts',(-16.8409895323044,-19.8997343347135,
-8.1482003364163));
#74255=CARTESIAN_POINT('Ctrl Pts',(-16.8188702864078,-19.8555532150832,
-8.14521743348146));
#74256=CARTESIAN_POINT('Ctrl Pts',(-16.7983237185206,-19.8106475457988,
-8.14223453054663));
#74257=CARTESIAN_POINT('Ctrl Pts',(-16.7793923012851,-19.765140666874,-8.1392516276118));
#74258=CARTESIAN_POINT('Ctrl Pts',(-16.7515419099038,-19.6981945754734,
-8.1348634186809));
#74259=CARTESIAN_POINT('Ctrl Pts',(-16.7270805292278,-19.6296853205151,
-8.13047520975));
#74260=CARTESIAN_POINT('Ctrl Pts',(-16.7061840240079,-19.5599896113515,
-8.12608700081911));
#74261=CARTESIAN_POINT('Ctrl Pts',(-16.6853185326665,-19.490397342176,-8.12170530471784));
#74262=CARTESIAN_POINT('Ctrl Pts',(-16.6680075510804,-19.4196225726488,
-8.11732360861658));
#74263=CARTESIAN_POINT('Ctrl Pts',(-16.6543788886961,-19.3480619060438,
-8.11294191251532));
#74264=CARTESIAN_POINT('Ctrl Pts',(-16.6407662410746,-19.276585328917,-8.10856536525568));
#74265=CARTESIAN_POINT('Ctrl Pts',(-16.6308274068039,-19.2043251607433,
-8.10418881799604));
#74266=CARTESIAN_POINT('Ctrl Pts',(-16.6246399100932,-19.1316914330408,
-8.0998122707364));
#74267=CARTESIAN_POINT('Ctrl Pts',(-16.618456337403,-19.0591037685929,-8.09543849901943));
#74268=CARTESIAN_POINT('Ctrl Pts',(-16.6160194227851,-18.9861434941228,
-8.09106472730246));
#74269=CARTESIAN_POINT('Ctrl Pts',(-16.6173550828665,-18.9132276545354,
-8.08669095558548));
#74270=CARTESIAN_POINT('Ctrl Pts',(-16.618690336502,-18.8403340034828,-8.08231851482193));
#74271=CARTESIAN_POINT('Ctrl Pts',(-16.6237958768595,-18.7674852424751,
-8.07794607405837));
#74272=CARTESIAN_POINT('Ctrl Pts',(-16.6326455110292,-18.6950986343316,
-8.07357363329481));
#74273=CARTESIAN_POINT('Ctrl Pts',(-16.641495371485,-18.6227101752548,-8.06920108072747));
#74274=CARTESIAN_POINT('Ctrl Pts',(-16.6540894553072,-18.5507843710743,
-8.06482852816014));
#74275=CARTESIAN_POINT('Ctrl Pts',(-16.6703498741218,-18.4797319003331,
-8.0604559755928));
#74276=CARTESIAN_POINT('Ctrl Pts',(-16.6866271686124,-18.4086056886577,
-8.05607888502548));
#74277=CARTESIAN_POINT('Ctrl Pts',(-16.7065782873147,-18.3383550912945,
-8.05170179445816));
#74278=CARTESIAN_POINT('Ctrl Pts',(-16.730074689432,-18.2693783261095,-8.04732470389083));
#74279=CARTESIAN_POINT('Ctrl Pts',(-16.7535839238066,-18.200363890153,-8.04294522283189));
#74280=CARTESIAN_POINT('Ctrl Pts',(-16.780642117511,-18.1326251197526,-8.03856574177295));
#74281=CARTESIAN_POINT('Ctrl Pts',(-16.8110725105121,-18.0665403057327,
-8.034186260714));
#74282=CARTESIAN_POINT('Ctrl Pts',(-16.8415568411806,-18.0003383568236,
-8.02979901705429));
#74283=CARTESIAN_POINT('Ctrl Pts',(-16.8754250830333,-17.9357966461506,
-8.02541177339457));
#74284=CARTESIAN_POINT('Ctrl Pts',(-16.9124547443358,-17.8732683922461,
-8.02102452973485));
#74285=CARTESIAN_POINT('Ctrl Pts',(-16.937631345852,-17.830755204799,-8.01804162680002));
#74286=CARTESIAN_POINT('Ctrl Pts',(-16.964268439743,-17.7891722056906,-8.0150587238652));
#74287=CARTESIAN_POINT('Ctrl Pts',(-16.992285306212,-17.7486218693016,-8.01207582093037));
#74288=CARTESIAN_POINT('Ctrl Pts',(-17.0335014860011,-17.6889674480278,
-8.00768761199947));
#74289=CARTESIAN_POINT('Ctrl Pts',(-17.0778664461833,-17.6313165376485,
-8.00329940306857));
#74290=CARTESIAN_POINT('Ctrl Pts',(-17.1251586260629,-17.5760209182156,
-7.99891119413767));
#74291=CARTESIAN_POINT('Ctrl Pts',(-17.1723806165064,-17.5208073666501,
-7.99452949803641));
#74292=CARTESIAN_POINT('Ctrl Pts',(-17.222520891325,-17.467942530263,-7.99014780193514));
#74293=CARTESIAN_POINT('Ctrl Pts',(-17.2753151507582,-17.4177485504024,
-7.98576610583387));
#74294=CARTESIAN_POINT('Ctrl Pts',(-17.3280473727351,-17.3676135524627,
-7.98138955857422));
#74295=CARTESIAN_POINT('Ctrl Pts',(-17.3834270362638,-17.3201435071857,
-7.97701301131459));
#74296=CARTESIAN_POINT('Ctrl Pts',(-17.4411513321106,-17.2756255424468,
-7.97263646405494));
#74297=CARTESIAN_POINT('Ctrl Pts',(-17.498839020048,-17.2311358103542,-7.96826269233796));
#74298=CARTESIAN_POINT('Ctrl Pts',(-17.5588680090007,-17.189594738041,-7.96388892062099));
#74299=CARTESIAN_POINT('Ctrl Pts',(-17.6209016583813,-17.1512498557863,
-7.95951514890401));
#74300=CARTESIAN_POINT('Ctrl Pts',(-17.682916430714,-17.112916642008,-7.95514270814045));
#74301=CARTESIAN_POINT('Ctrl Pts',(-17.7469342423164,-17.077777940832,-7.95077026737688));
#74302=CARTESIAN_POINT('Ctrl Pts',(-17.8125900634655,-17.0460375846162,
-7.94639782661332));
#74303=CARTESIAN_POINT('Ctrl Pts',(-17.8782475634413,-17.014296416796,-7.94202527404596));
#74304=CARTESIAN_POINT('Ctrl Pts',(-17.9455427209596,-16.9859539746113,
-7.9376527214786));
#74305=CARTESIAN_POINT('Ctrl Pts',(-18.0140880608572,-16.9611670587717,
-7.93328016891123));
#74306=CARTESIAN_POINT('Ctrl Pts',(-18.0827045396937,-16.9363544181361,
-7.9289030783439));
#74307=CARTESIAN_POINT('Ctrl Pts',(-18.1525733368288,-16.9151048356871,
-7.92452598777657));
#74308=CARTESIAN_POINT('Ctrl Pts',(-18.2232900373613,-16.8975257767347,
-7.92014889720925));
#74309=CARTESIAN_POINT('Ctrl Pts',(-18.2940453589085,-16.8799371172058,
-7.91576941615031));
#74310=CARTESIAN_POINT('Ctrl Pts',(-18.3656490319753,-16.866023064409,-7.91138993509137));
#74311=CARTESIAN_POINT('Ctrl Pts',(-18.4376872969909,-16.8558397527776,
-7.90701045403243));
#74312=CARTESIAN_POINT('Ctrl Pts',(-18.5098532493477,-16.8456383912947,
-7.9026232103727));
#74313=CARTESIAN_POINT('Ctrl Pts',(-18.5824548510295,-16.8391810190705,
-7.89823596671298));
#74314=CARTESIAN_POINT('Ctrl Pts',(-18.6550746705926,-16.8364717462587,
-7.89384872305326));
#74315=CARTESIAN_POINT('Ctrl Pts',(-18.7044491502656,-16.8346297018115,
-7.89086582011848));
#74316=CARTESIAN_POINT('Ctrl Pts',(-18.7538320255735,-16.834519193629,-7.8878829171837));
#74317=CARTESIAN_POINT('Ctrl Pts',(-18.8030934396838,-16.8361278165748,
-7.88490001424892));
#74318=CARTESIAN_POINT('Ctrl Pts',(-18.8755629038514,-16.8384942943756,
-7.88051180531802));
#74319=CARTESIAN_POINT('Ctrl Pts',(-18.9480521075246,-16.8445928606293,
-7.87612359638712));
#74320=CARTESIAN_POINT('Ctrl Pts',(-19.0201453327478,-16.8544276297237,
-7.87173538745623));
#74321=CARTESIAN_POINT('Ctrl Pts',(-19.0921315596717,-16.8642478023901,
-7.86735369135495));
#74322=CARTESIAN_POINT('Ctrl Pts',(-19.1637225008054,-16.8777931053666,
-7.86297199525368));
#74323=CARTESIAN_POINT('Ctrl Pts',(-19.2345042258077,-16.8950156733828,
-7.8585902991524));
#74324=CARTESIAN_POINT('Ctrl Pts',(-19.3052027766498,-16.912218003511,-7.85421375189277));
#74325=CARTESIAN_POINT('Ctrl Pts',(-19.3750935339399,-16.933088901349,-7.84983720463313));
#74326=CARTESIAN_POINT('Ctrl Pts',(-19.4437711636785,-16.9575291691252,
-7.8454606573735));
#74327=CARTESIAN_POINT('Ctrl Pts',(-19.5124052390626,-16.9819539372387,
-7.84108688565653));
#74328=CARTESIAN_POINT('Ctrl Pts',(-19.5798272600409,-17.0099434226001,
-7.83671311393956));
#74329=CARTESIAN_POINT('Ctrl Pts',(-19.6456468756563,-17.0413485471949,
-7.83233934222259));
#74330=CARTESIAN_POINT('Ctrl Pts',(-19.7114464621417,-17.0727441151049,
-7.82796690145903));
#74331=CARTESIAN_POINT('Ctrl Pts',(-19.7756441762372,-17.1075530511358,
-7.82359446069548));
#74332=CARTESIAN_POINT('Ctrl Pts',(-19.8378710435211,-17.145578753647,-7.81922201993193));
#74333=CARTESIAN_POINT('Ctrl Pts',(-19.900099501953,-17.1836054284797,-7.81484946736458));
#74334=CARTESIAN_POINT('Ctrl Pts',(-19.9603566029526,-17.2248487798652,
-7.81047691479722));
#74335=CARTESIAN_POINT('Ctrl Pts',(-20.0183007689805,-17.2690678757608,
-7.80610436222987));
#74336=CARTESIAN_POINT('Ctrl Pts',(-20.0763050716493,-17.3133328639019,
-7.80172727166255));
#74337=CARTESIAN_POINT('Ctrl Pts',(-20.1319912623922,-17.3605794693661,
-7.79735018109523));
#74338=CARTESIAN_POINT('Ctrl Pts',(-20.1850500777746,-17.4105258121556,
-7.79297309052791));
#74339=CARTESIAN_POINT('Ctrl Pts',(-20.2381378705453,-17.4604994324967,
-7.78859360946898));
#74340=CARTESIAN_POINT('Ctrl Pts',(-20.2885950971609,-17.5131753771409,
-7.78421412841004));
#74341=CARTESIAN_POINT('Ctrl Pts',(-20.3361505972381,-17.5682361242721,
-7.7798346473511));
#74342=CARTESIAN_POINT('Ctrl Pts',(-20.38379038912,-17.623394466208,-7.77544740369138));
#74343=CARTESIAN_POINT('Ctrl Pts',(-20.4285178872514,-17.6809456706585,
-7.77106016003166));
#74344=CARTESIAN_POINT('Ctrl Pts',(-20.4701036879201,-17.7405409685878,
-7.76667291637194));
#74345=CARTESIAN_POINT('Ctrl Pts',(-20.4983780251765,-17.7810600285903,
-7.76369001343712));
#74346=CARTESIAN_POINT('Ctrl Pts',(-20.5252009588539,-17.822523395732,-7.76070711050231));
#74347=CARTESIAN_POINT('Ctrl Pts',(-20.5505126306682,-17.864815166302,-7.7577242075675));
#74348=CARTESIAN_POINT('Ctrl Pts',(-20.5890325091508,-17.929175745687,-7.75318475796427));
#74349=CARTESIAN_POINT('Ctrl Pts',(-20.6241921153262,-17.9956925763863,
-7.74864530836104));
#74350=CARTESIAN_POINT('Ctrl Pts',(-20.6557527999575,-18.0639937073108,
-7.74410585875782));
#74351=CARTESIAN_POINT('Ctrl Pts',(-20.6876473131872,-18.1330172836155,
-7.73951839377987));
#74352=CARTESIAN_POINT('Ctrl Pts',(-20.7158660149379,-18.2038627902845,
-7.73493092880193));
#74353=CARTESIAN_POINT('Ctrl Pts',(-20.7402081049561,-18.2761168447072,
-7.73034346382399));
#74354=CARTESIAN_POINT('Ctrl Pts',(-20.7642010194568,-18.3473344496376,
-7.72582180381415));
#74355=CARTESIAN_POINT('Ctrl Pts',(-20.7844276391867,-18.4199200369922,
-7.72130014380432));
#74356=CARTESIAN_POINT('Ctrl Pts',(-20.8007427486143,-18.4934551155553,
-7.71677848379448));
#74357=CARTESIAN_POINT('Ctrl Pts',(-20.8174140154884,-18.5685954586084,
-7.71215811633248));
#74358=CARTESIAN_POINT('Ctrl Pts',(-20.8300007712016,-18.6447268210057,
-7.70753774887049));
#74359=CARTESIAN_POINT('Ctrl Pts',(-20.8384015048748,-18.7213849391716,
-7.70291738140849));
#74360=CARTESIAN_POINT('Ctrl Pts',(-20.8468022385479,-18.7980430573375,
-7.69829701394649));
#74361=CARTESIAN_POINT('Ctrl Pts',(-20.8510168371563,-18.8752274520633,
-7.6936766464845));
#74362=CARTESIAN_POINT('Ctrl Pts',(-20.850999949394,-18.9524628884561,-7.6890562790225));
#74363=CARTESIAN_POINT('Ctrl Pts',(-20.8476070359586,-18.9524685808987,
-7.68905589349203));
#74364=CARTESIAN_POINT('Ctrl Pts',(-20.8480883281253,-19.2000067147174,
-7.67422393751874));
#74365=CARTESIAN_POINT('Ctrl Pts',(-20.8073980344604,-19.4473941194524,
-7.65939198154544));
#74366=CARTESIAN_POINT('Ctrl Pts',(-20.7249098202513,-19.6789408942641,
-7.64456002557215));
#74367=CARTESIAN_POINT('Origin',(-18.734,-18.952,0.));
#74368=CARTESIAN_POINT('',(-20.7225805835101,-19.6781103655001,-6.84500601987795));
#74369=CARTESIAN_POINT('',(-20.7225805740154,-19.678110391503,-7.06814851970791));
#74370=CARTESIAN_POINT('',(-20.7225805821191,-19.6781103693095,0.));
#74371=CARTESIAN_POINT('',(-20.8510002457943,-18.9509645098827,-7.10922383901745));
#74372=CARTESIAN_POINT('Ctrl Pts',(-20.7225805740154,-19.678110391503,-7.06814851970791));
#74373=CARTESIAN_POINT('Ctrl Pts',(-20.746868289606,-19.6115942253996,-7.07222367278122));
#74374=CARTESIAN_POINT('Ctrl Pts',(-20.7678086356895,-19.5438870495728,
-7.07619430904908));
#74375=CARTESIAN_POINT('Ctrl Pts',(-20.829027411365,-19.3038845351043,-7.08986548609027));
#74376=CARTESIAN_POINT('Ctrl Pts',(-20.8510859889779,-19.1277568944903,
-7.0991404004068));
#74377=CARTESIAN_POINT('Ctrl Pts',(-20.8509997481143,-18.9509672928449,
-7.10922281586367));
#74378=CARTESIAN_POINT('Ctrl Pts',(-20.850999746731,-18.9509644609977,-7.10922297736565));
#74379=CARTESIAN_POINT('Ctrl Pts',(-20.8509866388502,-18.9241674207522,
-7.11075122973925));
#74380=CARTESIAN_POINT('Ctrl Pts',(-20.8504647357519,-18.8973740150214,
-7.11229817883972));
#74381=CARTESIAN_POINT('Ctrl Pts',(-20.8488772347217,-18.8561184486926,
-7.11471899714347));
#74382=CARTESIAN_POINT('Ctrl Pts',(-20.8481713903698,-18.8416446808493,
-7.11557568457049));
#74383=CARTESIAN_POINT('Ctrl Pts',(-20.8470399810025,-18.8224889222828,
-7.11672061828107));
#74384=CARTESIAN_POINT('Ctrl Pts',(-20.8467473096478,-18.8177990864489,
-7.11700181224313));
#74385=CARTESIAN_POINT('Ctrl Pts',(-20.8462061820977,-18.8095688211845,
-7.11749689627056));
#74386=CARTESIAN_POINT('Ctrl Pts',(-20.84596443064,-18.8060279489741,-7.11771041834802));
#74387=CARTESIAN_POINT('Ctrl Pts',(-20.8454718256639,-18.7990703880803,
-7.11813103347815));
#74388=CARTESIAN_POINT('Ctrl Pts',(-20.8452215797289,-18.7956536602765,
-7.11833809294867));
#74389=CARTESIAN_POINT('Ctrl Pts',(-20.844666932601,-18.7883250321715,-7.11878332283099));
#74390=CARTESIAN_POINT('Ctrl Pts',(-20.8443599504862,-18.7844133827758,
-7.11902163417546));
#74391=CARTESIAN_POINT('Ctrl Pts',(-20.8435234725859,-18.7741216578765,
-7.11965036568249));
#74392=CARTESIAN_POINT('Ctrl Pts',(-20.8429759117637,-18.7677431489571,
-7.12004177913951));
#74393=CARTESIAN_POINT('Ctrl Pts',(-20.8405832036317,-18.7412797723747,
-7.12167265453771));
#74394=CARTESIAN_POINT('Ctrl Pts',(-20.8384800666777,-18.7212200432533,
-7.12292554864206));
#74395=CARTESIAN_POINT('Ctrl Pts',(-20.8355857385863,-18.6969616625413,
-7.12445842633881));
#74396=CARTESIAN_POINT('Ctrl Pts',(-20.8350679540685,-18.6927305995594,
-7.12472644129594));
#74397=CARTESIAN_POINT('Ctrl Pts',(-20.8313092275801,-18.662767106493,-7.12662898074645));
#74398=CARTESIAN_POINT('Ctrl Pts',(-20.8276085513941,-18.6370955961657,
-7.12828257683198));
#74399=CARTESIAN_POINT('Ctrl Pts',(-20.7949897013469,-18.436934131115,-7.14132865003135));
#74400=CARTESIAN_POINT('Ctrl Pts',(-20.7447788267489,-18.2666183148405,
-7.15326722317378));
#74401=CARTESIAN_POINT('Ctrl Pts',(-20.650345255995,-18.0504506566882,-7.16847632404371));
#74402=CARTESIAN_POINT('Ctrl Pts',(-20.6244734804001,-17.9973894131658,
-7.17222246512559));
#74403=CARTESIAN_POINT('Ctrl Pts',(-20.5792806416933,-17.9137672016062,
-7.17813934634324));
#74404=CARTESIAN_POINT('Ctrl Pts',(-20.5613370651451,-17.8825012897303,
-7.18035501009081));
#74405=CARTESIAN_POINT('Ctrl Pts',(-20.536883982782,-17.8423066085726,-7.18320968006345));
#74406=CARTESIAN_POINT('Ctrl Pts',(-20.5310916875033,-17.8329506033169,
-7.18387462150893));
#74407=CARTESIAN_POINT('Ctrl Pts',(-20.5215271011513,-17.8177672023027,
-7.18495461053093));
#74408=CARTESIAN_POINT('Ctrl Pts',(-20.5177986866752,-17.811912536722,-7.1853712685657));
#74409=CARTESIAN_POINT('Ctrl Pts',(-20.5105552822049,-17.8006608624826,
-7.18617247903258));
#74410=CARTESIAN_POINT('Ctrl Pts',(-20.507044329755,-17.7952613577613,-7.18655717563589));
#74411=CARTESIAN_POINT('Ctrl Pts',(-20.4989233190818,-17.7828958759464,
-7.18743869924245));
#74412=CARTESIAN_POINT('Ctrl Pts',(-20.4942965442247,-17.7759409646788,
-7.18793489340288));
#74413=CARTESIAN_POINT('Ctrl Pts',(-20.4818382944251,-17.7574521134627,
-7.18925512890039));
#74414=CARTESIAN_POINT('Ctrl Pts',(-20.473933765784,-17.7459677196544,-7.19007640843862));
#74415=CARTESIAN_POINT('Ctrl Pts',(-20.4094922514753,-17.6542938047509,
-7.1966441130327));
#74416=CARTESIAN_POINT('Ctrl Pts',(-20.3475528107261,-17.578039846708,-7.20217270330802));
#74417=CARTESIAN_POINT('Ctrl Pts',(-20.1871361598569,-17.4064279507383,
-7.21512831208192));
#74418=CARTESIAN_POINT('Ctrl Pts',(-20.0842734926071,-17.3157980809827,
-7.22240524090073));
#74419=CARTESIAN_POINT('Ctrl Pts',(-19.9317674131666,-17.2056671649268,
-7.23282860991743));
#74420=CARTESIAN_POINT('Ctrl Pts',(-19.8890657264697,-17.1771344824893,
-7.23571524646854));
#74421=CARTESIAN_POINT('Ctrl Pts',(-19.8300448816548,-17.1407300237036,
-7.23972171332931));
#74422=CARTESIAN_POINT('Ctrl Pts',(-19.8145979528711,-17.1314722386223,
-7.24077179125907));
#74423=CARTESIAN_POINT('Ctrl Pts',(-19.7915652683004,-17.1180645010709,
-7.24234261682033));
#74424=CARTESIAN_POINT('Ctrl Pts',(-19.784068779426,-17.1137619131528,-7.24285465988697));
#74425=CARTESIAN_POINT('Ctrl Pts',(-19.7704483273461,-17.1060549966457,
-7.24378679889659));
#74426=CARTESIAN_POINT('Ctrl Pts',(-19.7643333689349,-17.1026349099216,
-7.24420593845753));
#74427=CARTESIAN_POINT('Ctrl Pts',(-19.7546719209946,-17.0972940675338,
-7.24486937067347));
#74428=CARTESIAN_POINT('Ctrl Pts',(-19.7511366636923,-17.0953529487323,
-7.24511238230894));
#74429=CARTESIAN_POINT('Ctrl Pts',(-19.7475868213506,-17.0934170032813,
-7.24535667124713));
#74430=CARTESIAN_POINT('Ctrl Pts',(-19.7475777274738,-17.0934120439225,
-7.24535729706082));
#74431=CARTESIAN_POINT('Ctrl Pts',(-19.7475594840348,-17.0934020950104,
-7.24535855252391));
#74432=CARTESIAN_POINT('Ctrl Pts',(-19.7475503350351,-17.093397105765,-7.24535918213463));
#74433=CARTESIAN_POINT('Ctrl Pts',(-19.7475319812136,-17.0933870970083,
-7.24536044520128));
#74434=CARTESIAN_POINT('Ctrl Pts',(-19.7475227762295,-17.0933820774097,
-7.24536107866839));
#74435=CARTESIAN_POINT('Ctrl Pts',(-19.7475043103821,-17.0933720079187,
-7.24536234945181));
#74436=CARTESIAN_POINT('Ctrl Pts',(-19.7474950492077,-17.0933669578578,
-7.24536298678955));
#74437=CARTESIAN_POINT('Ctrl Pts',(-19.7474764703428,-17.0933568270983,
-7.24536426535814));
#74438=CARTESIAN_POINT('Ctrl Pts',(-19.7474671527697,-17.0933517464648,
-7.24536490658093));
#74439=CARTESIAN_POINT('Ctrl Pts',(-19.7474484608541,-17.0933415544252,
-7.24536619293709));
#74440=CARTESIAN_POINT('Ctrl Pts',(-19.7474390861883,-17.093336442844,-7.24536683809274));
#74441=CARTESIAN_POINT('Ctrl Pts',(-19.7474202797423,-17.0933261887242,
-7.24536813233846));
#74442=CARTESIAN_POINT('Ctrl Pts',(-19.7474108477663,-17.09332104608,-7.24536878144202));
#74443=CARTESIAN_POINT('Ctrl Pts',(-19.747391926084,-17.0933107295019,-7.24537008362602));
#74444=CARTESIAN_POINT('Ctrl Pts',(-19.7473824364263,-17.0933055555957,
-7.24537073670312));
#74445=CARTESIAN_POINT('Ctrl Pts',(-19.7473633987774,-17.0932951761679,
-7.2453720468758));
#74446=CARTESIAN_POINT('Ctrl Pts',(-19.7473538509974,-17.0932899707628,
-7.24537270395685));
#74447=CARTESIAN_POINT('Ctrl Pts',(-19.7473346966567,-17.093279528097,-7.24537402216826));
#74448=CARTESIAN_POINT('Ctrl Pts',(-19.747325090272,-17.0932742909334,-7.24537468328653));
#74449=CARTESIAN_POINT('Ctrl Pts',(-19.747305818564,-17.0932637846683,-7.24537600958331));
#74450=CARTESIAN_POINT('Ctrl Pts',(-19.7472961530412,-17.0932585154592,
-7.24537667477558));
#74451=CARTESIAN_POINT('Ctrl Pts',(-19.747276762527,-17.0932479448174,-7.24537800925691));
#74452=CARTESIAN_POINT('Ctrl Pts',(-19.7472670376847,-17.0932426434673,
-7.24537867853574));
#74453=CARTESIAN_POINT('Ctrl Pts',(-19.7472475657517,-17.093232028837,-7.2453800186287));
#74454=CARTESIAN_POINT('Ctrl Pts',(-19.7472377621061,-17.0932266847277,
-7.24538069333527));
#74455=CARTESIAN_POINT('Ctrl Pts',(-19.7472181122366,-17.0932159735023,
-7.24538204568256));
#74456=CARTESIAN_POINT('Ctrl Pts',(-19.7472082678274,-17.0932106073755,
-7.24538272319859));
#74457=CARTESIAN_POINT('Ctrl Pts',(-19.7471885165869,-17.0931998412995,
-7.24538408253095));
#74458=CARTESIAN_POINT('Ctrl Pts',(-19.7471786113506,-17.0931944422209,
-7.24538476423753));
#74459=CARTESIAN_POINT('Ctrl Pts',(-19.7471587045236,-17.0931835917501,
-7.2453861342864));
#74460=CARTESIAN_POINT('Ctrl Pts',(-19.7471487549029,-17.0931781686866,
-7.24538681905178));
#74461=CARTESIAN_POINT('Ctrl Pts',(-19.7441393580398,-17.0915379211943,
-7.2455939362838));
#74462=CARTESIAN_POINT('Ctrl Pts',(-19.7411360224105,-17.0899103939135,
-7.24580083676566));
#74463=CARTESIAN_POINT('Ctrl Pts',(-19.734094710212,-17.0861166788207,-7.24628637285296));
#74464=CARTESIAN_POINT('Ctrl Pts',(-19.730053643727,-17.0839563346765,-7.2465653748392));
#74465=CARTESIAN_POINT('Ctrl Pts',(-19.7176093263313,-17.0773554933554,
-7.24742554672184));
#74466=CARTESIAN_POINT('Ctrl Pts',(-19.7091832947715,-17.0729585244077,
-7.24800935846962));
#74467=CARTESIAN_POINT('Ctrl Pts',(-19.5939326404601,-17.0138010722072,
-7.25601063328275));
#74468=CARTESIAN_POINT('Ctrl Pts',(-19.482680090488,-16.9681727197242,-7.2639085184497));
#74469=CARTESIAN_POINT('Ctrl Pts',(-19.2643432133411,-16.8996186070641,
-7.27902715286637));
#74470=CARTESIAN_POINT('Ctrl Pts',(-19.158142028617,-16.8750694943601,-7.28622009168223));
#74471=CARTESIAN_POINT('Ctrl Pts',(-18.9765362974362,-16.847608501746,-7.29801960758239));
#74472=CARTESIAN_POINT('Ctrl Pts',(-18.9020074916349,-16.8403506339402,
-7.30272662723546));
#74473=CARTESIAN_POINT('Ctrl Pts',(-18.8084824368351,-16.8362273237884,
-7.30846140055924));
#74474=CARTESIAN_POINT('Ctrl Pts',(-18.7897110327954,-16.835649847663,-7.30960397013258));
#74475=CARTESIAN_POINT('Ctrl Pts',(-18.7623861790448,-16.8351730558821,
-7.31125530604847));
#74476=CARTESIAN_POINT('Ctrl Pts',(-18.753837494632,-16.835075683058,-7.31177024611993));
#74477=CARTESIAN_POINT('Ctrl Pts',(-18.7388400531612,-16.8349957119377,
-7.31267074275303));
#74478=CARTESIAN_POINT('Ctrl Pts',(-18.7323915726135,-16.8349907897751,
-7.31305699344597));
#74479=CARTESIAN_POINT('Ctrl Pts',(-18.7198640355442,-16.8350384674625,
-7.31380558151473));
#74480=CARTESIAN_POINT('Ctrl Pts',(-18.7137850364791,-16.8350877882703,
-7.31416801775506));
#74481=CARTESIAN_POINT('Ctrl Pts',(-18.6992436604134,-16.8352684100428,
-7.31503307664059));
#74482=CARTESIAN_POINT('Ctrl Pts',(-18.690781650748,-16.8354242738534,-7.31553492693704));
#74483=CARTESIAN_POINT('Ctrl Pts',(-18.6601926562498,-16.8361712217935,
-7.31734362593767));
#74484=CARTESIAN_POINT('Ctrl Pts',(-18.6380738560968,-16.8370585889712,
-7.31864121513094));
#74485=CARTESIAN_POINT('Ctrl Pts',(-18.4309382179136,-16.8486248645878,
-7.33070667458507));
#74486=CARTESIAN_POINT('Ctrl Pts',(-18.2480668271197,-16.8832060533965,
-7.34062083838386));
#74487=CARTESIAN_POINT('Ctrl Pts',(-17.9957351896204,-16.9662748173921,
-7.35510190619751));
#74488=CARTESIAN_POINT('Ctrl Pts',(-17.9209448170173,-16.9957079245597,
-7.35951815846977));
#74489=CARTESIAN_POINT('Ctrl Pts',(-17.8152483351737,-17.0444135928366,
-7.36617480174179));
#74490=CARTESIAN_POINT('Ctrl Pts',(-17.7828765934529,-17.0603461103899,
-7.36827316987093));
#74491=CARTESIAN_POINT('Ctrl Pts',(-17.7443150231686,-17.0805651404608,
-7.37086431307254));
#74492=CARTESIAN_POINT('Ctrl Pts',(-17.7377186261131,-17.0840684682947,
-7.37131085341731));
#74493=CARTESIAN_POINT('Ctrl Pts',(-17.7274774565254,-17.089577203062,-7.37200948613473));
#74494=CARTESIAN_POINT('Ctrl Pts',(-17.72381974778,-17.091558610862,-7.37226007914074));
#74495=CARTESIAN_POINT('Ctrl Pts',(-17.7170375932739,-17.0952584513303,
-7.37272676780927));
#74496=CARTESIAN_POINT('Ctrl Pts',(-17.7139116406221,-17.0969740018784,
-7.37294267966426));
#74497=CARTESIAN_POINT('Ctrl Pts',(-17.7068420605829,-17.1008771231945,
-7.37343281451122));
#74498=CARTESIAN_POINT('Ctrl Pts',(-17.702901100051,-17.1030693914606,-7.37370733474758));
#74499=CARTESIAN_POINT('Ctrl Pts',(-17.6927446607421,-17.1087617620941,
-7.3744180977834));
#74500=CARTESIAN_POINT('Ctrl Pts',(-17.6865398720474,-17.1122806843829,
-7.37485550627048));
#74501=CARTESIAN_POINT('Ctrl Pts',(-17.6485646925553,-17.134071939506,-7.37755163874075));
#74502=CARTESIAN_POINT('Ctrl Pts',(-17.6172574934826,-17.1531342349018,
-7.37985651015451));
#74503=CARTESIAN_POINT('Ctrl Pts',(-17.4431946581303,-17.2654126553866,
-7.39307508997707));
#74504=CARTESIAN_POINT('Ctrl Pts',(-17.3116151507582,-17.3747936954772,
-7.40457887290739));
#74505=CARTESIAN_POINT('Ctrl Pts',(-17.1290716563344,-17.568164802461,-7.4218605509172));
#74506=CARTESIAN_POINT('Ctrl Pts',(-17.06832692473,-17.6419113369407,-7.42792345417126));
#74507=CARTESIAN_POINT('Ctrl Pts',(-17.0003026282046,-17.7369114330647,
-7.4351006451469));
#74508=CARTESIAN_POINT('Ctrl Pts',(-16.9881101287382,-17.7544961742685,
-7.43640483688866));
#74509=CARTESIAN_POINT('Ctrl Pts',(-16.9711646351047,-17.7797450502855,
-7.43824384141809));
#74510=CARTESIAN_POINT('Ctrl Pts',(-16.9661910750996,-17.7872589129673,
-7.4387869668367));
#74511=CARTESIAN_POINT('Ctrl Pts',(-16.9576980652593,-17.8002695490169,
-7.43972037008653));
#74512=CARTESIAN_POINT('Ctrl Pts',(-16.9541558127354,-17.805751220011,-7.44011149910188));
#74513=CARTESIAN_POINT('Ctrl Pts',(-16.9474249306634,-17.8162737577625,
-7.44085826804866));
#74514=CARTESIAN_POINT('Ctrl Pts',(-16.9442321496843,-17.8213118826221,
-7.44121406002586));
#74515=CARTESIAN_POINT('Ctrl Pts',(-16.9359915233256,-17.8344377386945,
-7.44213649720445));
#74516=CARTESIAN_POINT('Ctrl Pts',(-16.9309769064983,-17.8425462520201,
-7.44270191117853));
#74517=CARTESIAN_POINT('Ctrl Pts',(-16.9140962511439,-17.8702586059278,
-7.4446195765534));
#74518=CARTESIAN_POINT('Ctrl Pts',(-16.9024935405953,-17.8900215405943,
-7.44596221069099));
#74519=CARTESIAN_POINT('Ctrl Pts',(-16.8043405028427,-18.0636009964475,
-7.45755042631187));
#74520=CARTESIAN_POINT('Ctrl Pts',(-16.7370196429506,-18.2274900491444,
-7.46703498002691));
#74521=CARTESIAN_POINT('Ctrl Pts',(-16.6682260941955,-18.4811345108922,
-7.48133695378272));
#74522=CARTESIAN_POINT('Ctrl Pts',(-16.6507522877699,-18.5657193323404,
-7.48606346403716));
#74523=CARTESIAN_POINT('Ctrl Pts',(-16.6331395152954,-18.6883880526693,
-7.49314030236153));
#74524=CARTESIAN_POINT('Ctrl Pts',(-16.6287846908924,-18.7257829729442,
-7.49532720628924));
#74525=CARTESIAN_POINT('Ctrl Pts',(-16.6247551783058,-18.7708027119098,
-7.49801652806066));
#74526=CARTESIAN_POINT('Ctrl Pts',(-16.6241214512125,-18.77833745219,-7.4984685224453));
#74527=CARTESIAN_POINT('Ctrl Pts',(-16.6232000990504,-18.7900424412373,
-7.4991738467582));
#74528=CARTESIAN_POINT('Ctrl Pts',(-16.6228844304726,-18.79421050702,-7.49942563050811));
#74529=CARTESIAN_POINT('Ctrl Pts',(-16.622322490706,-18.8019340189597,-7.49989338918839));
#74530=CARTESIAN_POINT('Ctrl Pts',(-16.6220728526338,-18.8054891623207,
-7.50010917304562));
#74531=CARTESIAN_POINT('Ctrl Pts',(-16.6215294670781,-18.8135177086928,
-7.50059754107513));
#74532=CARTESIAN_POINT('Ctrl Pts',(-16.6212409528226,-18.8179913988441,
-7.50087041330138));
#74533=CARTESIAN_POINT('Ctrl Pts',(-16.6204331437055,-18.8311688394999,
-7.50167628804254));
#74534=CARTESIAN_POINT('Ctrl Pts',(-16.6199534162411,-18.8398747973703,
-7.502211426756));
#74535=CARTESIAN_POINT('Ctrl Pts',(-16.6169219287903,-18.9018570173764,
-7.50603952088913));
#74536=CARTESIAN_POINT('Ctrl Pts',(-16.6163308645768,-18.9552055382128,
-7.50942951252395));
#74537=CARTESIAN_POINT('Ctrl Pts',(-16.6182285227753,-19.0262657143222,
-7.51402367808511));
#74538=CARTESIAN_POINT('Ctrl Pts',(-16.6189259022126,-19.0440101961314,
-7.51517747973296));
#74539=CARTESIAN_POINT('Ctrl Pts',(-16.6223540538807,-19.1100518571353,
-7.51949180158957));
#74540=CARTESIAN_POINT('Ctrl Pts',(-16.6265166660615,-19.1582589459159,
-7.52268074662665));
#74541=CARTESIAN_POINT('Ctrl Pts',(-16.6454648144414,-19.3148691955398,
-7.5331014298174));
#74542=CARTESIAN_POINT('Ctrl Pts',(-16.6670001823719,-19.4222855452956,
-7.54033412189648));
#74543=CARTESIAN_POINT('Ctrl Pts',(-16.711722965055,-19.5805861668141,-7.55090754546354));
#74544=CARTESIAN_POINT('Ctrl Pts',(-16.7287685493419,-19.6330085355309,
-7.55439665486008));
#74545=CARTESIAN_POINT('Ctrl Pts',(-16.7597140585279,-19.7168926158931,
-7.5599541857702));
#74546=CARTESIAN_POINT('Ctrl Pts',(-16.7723675331868,-19.748783517653,-7.56206104536376));
#74547=CARTESIAN_POINT('Ctrl Pts',(-16.7900202527158,-19.7903009984069,
-7.56479756735056));
#74548=CARTESIAN_POINT('Ctrl Pts',(-16.7943256150807,-19.8002152492467,
-7.5654505709248));
#74549=CARTESIAN_POINT('Ctrl Pts',(-16.801502790366,-19.8164021733181,-7.56651606950218));
#74550=CARTESIAN_POINT('Ctrl Pts',(-16.8043296294835,-19.8226944615553,
-7.56693009394265));
#74551=CARTESIAN_POINT('Ctrl Pts',(-16.8098619204464,-19.8348495569959,
-7.56772960894873));
#74552=CARTESIAN_POINT('Ctrl Pts',(-16.8125635355261,-19.840714016932,-7.56811522585636));
#74553=CARTESIAN_POINT('Ctrl Pts',(-16.8188645805864,-19.8542287992774,
-7.56900364654562));
#74554=CARTESIAN_POINT('Ctrl Pts',(-16.8224831099357,-19.8618701352942,
-7.56950578426038));
#74555=CARTESIAN_POINT('Ctrl Pts',(-16.8323404327509,-19.8823677167773,
-7.5708523952996));
#74556=CARTESIAN_POINT('Ctrl Pts',(-16.8386638468601,-19.8951829513108,
-7.57169392720912));
#74557=CARTESIAN_POINT('Ctrl Pts',(-16.8978743785234,-20.0121804172648,
-7.57937578355708));
#74558=CARTESIAN_POINT('Ctrl Pts',(-16.959174384457,-20.1118875431223,-7.58589942217557));
#74559=CARTESIAN_POINT('Ctrl Pts',(-17.1248260473085,-20.3371885100922,
-7.60120841485988));
#74560=CARTESIAN_POINT('Ctrl Pts',(-17.2360472925864,-20.4567637133646,
-7.60981056431433));
#74561=CARTESIAN_POINT('Ctrl Pts',(-17.384542851605,-20.583474198908,-7.62101974207945));
#74562=CARTESIAN_POINT('Ctrl Pts',(-17.4097150985187,-20.6039721234287,
-7.62291303699605));
#74563=CARTESIAN_POINT('Ctrl Pts',(-17.441061810619,-20.6283210320993,-7.62527637617195));
#74564=CARTESIAN_POINT('Ctrl Pts',(-17.4467992531642,-20.6327306738812,
-7.62570916793069));
#74565=CARTESIAN_POINT('Ctrl Pts',(-17.4558297968618,-20.6395979424802,
-7.62639091787312));
#74566=CARTESIAN_POINT('Ctrl Pts',(-17.4591076999722,-20.6420755918964,
-7.6266384918909));
#74567=CARTESIAN_POINT('Ctrl Pts',(-17.4652486200129,-20.6466892621697,
-7.62710255766595));
#74568=CARTESIAN_POINT('Ctrl Pts',(-17.4681098369447,-20.6488275852177,
-7.62731888432482));
#74569=CARTESIAN_POINT('Ctrl Pts',(-17.474654132372,-20.6536926825989,-7.62781390872651));
#74570=CARTESIAN_POINT('Ctrl Pts',(-17.478340648725,-20.6564147361972,-7.6280929287195));
#74571=CARTESIAN_POINT('Ctrl Pts',(-17.4897013524436,-20.6647464018606,
-7.62895321007945));
#74572=CARTESIAN_POINT('Ctrl Pts',(-17.4974043847981,-20.6703162218043,
-7.62953711425411));
#74573=CARTESIAN_POINT('Ctrl Pts',(-17.6024905108618,-20.7452281187138,
-7.63750797473245));
#74574=CARTESIAN_POINT('Ctrl Pts',(-17.7055287611058,-20.8062440750724,
-7.64537152959528));
#74575=CARTESIAN_POINT('Ctrl Pts',(-17.9113004362447,-20.9056468486291,
-7.66046832742099));
#74576=CARTESIAN_POINT('Ctrl Pts',(-18.0129739427331,-20.9454130233632,
-7.66767364089163));
#74577=CARTESIAN_POINT('Ctrl Pts',(-18.1890958317102,-20.9990483206543,
-7.67950324040887));
#74578=CARTESIAN_POINT('Ctrl Pts',(-18.2620468182198,-21.0170883091843,
-7.68422764383675));
#74579=CARTESIAN_POINT('Ctrl Pts',(-18.3542890648221,-21.0347536132033,
-7.6899811799499));
#74580=CARTESIAN_POINT('Ctrl Pts',(-18.3728151392171,-21.0380461499747,
-7.69112597537445));
#74581=CARTESIAN_POINT('Ctrl Pts',(-18.3998260415797,-21.0424760141134,
-7.69277991515912));
#74582=CARTESIAN_POINT('Ctrl Pts',(-18.4082773660338,-21.0438094963808,
-7.6932952606614));
#74583=CARTESIAN_POINT('Ctrl Pts',(-18.4231132223346,-21.0460582624343,
-7.69419622489128));
#74584=CARTESIAN_POINT('Ctrl Pts',(-18.4294942417659,-21.0469956657775,
-7.69458253997317));
#74585=CARTESIAN_POINT('Ctrl Pts',(-18.4418961018197,-21.0487597011936,
-7.6953310776126));
#74586=CARTESIAN_POINT('Ctrl Pts',(-18.4479164077418,-21.0495895955375,
-7.69569339985829));
#74587=CARTESIAN_POINT('Ctrl Pts',(-18.4623217801259,-21.051512192436,-7.69655790776223));
#74588=CARTESIAN_POINT('Ctrl Pts',(-18.4707100252494,-21.0525806087103,
-7.6970593233283));
#74589=CARTESIAN_POINT('Ctrl Pts',(-18.5010310085101,-21.0562581332465,
-7.69886480164759));
#74590=CARTESIAN_POINT('Ctrl Pts',(-18.5229983294144,-21.0585742786541,
-7.70015964857557));
#74591=CARTESIAN_POINT('Ctrl Pts',(-18.7300515698798,-21.0771336873533,
-7.7122504139795));
#74592=CARTESIAN_POINT('Ctrl Pts',(-18.9164774519554,-21.0692899551196,
-7.72218745783808));
#74593=CARTESIAN_POINT('Ctrl Pts',(-19.2071139739458,-21.0183468027605,
-7.73827355701547));
#74594=CARTESIAN_POINT('Ctrl Pts',(-19.313094178067,-20.9911835347628,-7.74429703988687));
#74595=CARTESIAN_POINT('Ctrl Pts',(-19.4276559444185,-20.9521673888345,
-7.75144017293873));
#74596=CARTESIAN_POINT('Ctrl Pts',(-19.4387901513323,-20.9482712693633,
-7.75214127981236));
#74597=CARTESIAN_POINT('Ctrl Pts',(-19.4545996008962,-20.942590427378,-7.75314736748704));
#74598=CARTESIAN_POINT('Ctrl Pts',(-19.4593022049987,-20.9408817824684,
-7.75344797508748));
#74599=CARTESIAN_POINT('Ctrl Pts',(-19.4674062068257,-20.9379047092452,
-7.75396840202993));
#74600=CARTESIAN_POINT('Ctrl Pts',(-19.4708105153217,-20.9366441602408,
-7.75418775233713));
#74601=CARTESIAN_POINT('Ctrl Pts',(-19.4774131010705,-20.9341800217499,
-7.75461462403103));
#74602=CARTESIAN_POINT('Ctrl Pts',(-19.4806117122579,-20.9329774426284,
-7.75482207911996));
#74603=CARTESIAN_POINT('Ctrl Pts',(-19.489251472756,-20.9297052617764,-7.75538418810968));
#74604=CARTESIAN_POINT('Ctrl Pts',(-19.4946869725986,-20.9276209700844,
-7.75573970867091));
#74605=CARTESIAN_POINT('Ctrl Pts',(-19.5149316906852,-20.9197620169374,
-7.75707070697389));
#74606=CARTESIAN_POINT('Ctrl Pts',(-19.5296838931936,-20.9138432068835,
-7.75805430571519));
#74607=CARTESIAN_POINT('Ctrl Pts',(-19.6585815730293,-20.860434534178,-7.76676058775287));
#74608=CARTESIAN_POINT('Ctrl Pts',(-19.768419834445,-20.8032005102041,-7.77494143333174));
#74609=CARTESIAN_POINT('Ctrl Pts',(-20.0135308825098,-20.6468230523889,
-7.79415453954332));
#74610=CARTESIAN_POINT('Ctrl Pts',(-20.1433214528168,-20.540539676929,-7.80507087500697));
#74611=CARTESIAN_POINT('Ctrl Pts',(-20.2740377425466,-20.404730611505,-7.81664823128841));
#74612=CARTESIAN_POINT('Ctrl Pts',(-20.2885732390007,-20.3891654653027,
-7.81794616042519));
#74613=CARTESIAN_POINT('Ctrl Pts',(-20.308910170494,-20.3667182890134,-7.81977794443242));
#74614=CARTESIAN_POINT('Ctrl Pts',(-20.3149060462295,-20.3600149002377,
-7.82032002345927));
#74615=CARTESIAN_POINT('Ctrl Pts',(-20.3251770157455,-20.3483836360491,
-7.82125219272436));
#74616=CARTESIAN_POINT('Ctrl Pts',(-20.3294723482453,-20.3434738739644,
-7.82164312821546));
#74617=CARTESIAN_POINT('Ctrl Pts',(-20.3376538037636,-20.3340344047315,
-7.82238991155202));
#74618=CARTESIAN_POINT('Ctrl Pts',(-20.3415435938569,-20.3295079720858,
-7.82274590959635));
#74619=CARTESIAN_POINT('Ctrl Pts',(-20.3516099372605,-20.3176933609615,
-7.82366971094577));
#74620=CARTESIAN_POINT('Ctrl Pts',(-20.3577564351206,-20.3103796631465,
-7.82423627564897));
#74621=CARTESIAN_POINT('Ctrl Pts',(-20.3785535031676,-20.2852904294535,
-7.82616210536949));
#74622=CARTESIAN_POINT('Ctrl Pts',(-20.392963695283,-20.2673171150141,-7.82751163975618));
#74623=CARTESIAN_POINT('Ctrl Pts',(-20.5142337192113,-20.1108971021652,
-7.83901216327063));
#74624=CARTESIAN_POINT('Ctrl Pts',(-20.6038499556641,-19.9599397095911,
-7.84841819641638));
#74625=CARTESIAN_POINT('Ctrl Pts',(-20.6913707348718,-19.759648453698,-7.86031013461783));
#74626=CARTESIAN_POINT('Ctrl Pts',(-20.7076099334921,-19.7191101143336,
-7.86269371541934));
#74627=CARTESIAN_POINT('Ctrl Pts',(-20.7225805730004,-19.6781103942827,
-7.86510594064261));
#74628=CARTESIAN_POINT('',(-20.8523539331562,-18.9537405760439,-6.88905704666127));
#74629=CARTESIAN_POINT('Ctrl Pts',(-20.7249098202513,-19.6789408942641,
-7.64456002557215));
#74630=CARTESIAN_POINT('Ctrl Pts',(-20.6989345116989,-19.7518543277492,
-7.63988948401012));
#74631=CARTESIAN_POINT('Ctrl Pts',(-20.3954318373018,-20.4707351797969,
-7.59282700688761));
#74632=CARTESIAN_POINT('Ctrl Pts',(-19.0148744683191,-21.4394564387197,
-7.50337259420462));
#74633=CARTESIAN_POINT('Ctrl Pts',(-16.794474806048,-20.5345839704445,-7.3761967875232));
#74634=CARTESIAN_POINT('Ctrl Pts',(-16.3534691287178,-18.1777889355253,
-7.24902098084176));
#74635=CARTESIAN_POINT('Ctrl Pts',(-18.0964527733798,-16.5312844993037,
-7.12184517416032));
#74636=CARTESIAN_POINT('Ctrl Pts',(-20.292776587038,-17.0731745935747,-7.00185719610017));
#74637=CARTESIAN_POINT('Ctrl Pts',(-20.8471439801893,-18.3695361434103,
-6.92426115360048));
#74638=CARTESIAN_POINT('Ctrl Pts',(-20.8523539331563,-18.9537405760439,
-6.88905704666127));
#74639=CARTESIAN_POINT('Ctrl Pts',(-20.8509992391743,-18.9537948079469,
-6.88983562681212));
#74640=CARTESIAN_POINT('Ctrl Pts',(-20.8509308803788,-19.0344248933761,
-6.88542680327367));
#74641=CARTESIAN_POINT('Ctrl Pts',(-20.846256125498,-19.1149800327588,-6.88096325172215));
#74642=CARTESIAN_POINT('Ctrl Pts',(-20.8342751935892,-19.2186387282606,
-6.87493021363211));
#74643=CARTESIAN_POINT('Ctrl Pts',(-20.8311546068468,-19.2421629736403,
-6.87354147870167));
#74644=CARTESIAN_POINT('Ctrl Pts',(-20.8267567240817,-19.2715211958718,
-6.87177823640636));
#74645=CARTESIAN_POINT('Ctrl Pts',(-20.8258491613927,-19.2774098721672,
-6.87142304382925));
#74646=CARTESIAN_POINT('Ctrl Pts',(-20.8242842192338,-19.2872867738242,
-6.87082461715517));
#74647=CARTESIAN_POINT('Ctrl Pts',(-20.8236402480805,-19.2912771298949,
-6.87058211407328));
#74648=CARTESIAN_POINT('Ctrl Pts',(-20.8224405316354,-19.2985781517168,
-6.87013703098857));
#74649=CARTESIAN_POINT('Ctrl Pts',(-20.8218883299891,-19.3018893976088,
-6.8699346501367));
#74650=CARTESIAN_POINT('Ctrl Pts',(-20.82073183337,-19.3087240321801,-6.86951581921289));
#74651=CARTESIAN_POINT('Ctrl Pts',(-20.8201264940706,-19.312247178472,-6.86929930838652));
#74652=CARTESIAN_POINT('Ctrl Pts',(-20.8187199416278,-19.3203110438727,
-6.86880236553774));
#74653=CARTESIAN_POINT('Ctrl Pts',(-20.8179128178603,-19.3248506761268,
-6.86852160159985));
#74654=CARTESIAN_POINT('Ctrl Pts',(-20.8153705417999,-19.338883443171,-6.86765067971333));
#74655=CARTESIAN_POINT('Ctrl Pts',(-20.8135853308845,-19.3483672215856,
-6.8670577851907));
#74656=CARTESIAN_POINT('Ctrl Pts',(-20.7945684251442,-19.445726446506,-6.86092929323585));
#74657=CARTESIAN_POINT('Ctrl Pts',(-20.7718441164442,-19.5324271271654,
-6.85512345423274));
#74658=CARTESIAN_POINT('Ctrl Pts',(-20.7369695611002,-19.6377557279032,
-6.84783205872112));
#74659=CARTESIAN_POINT('Ctrl Pts',(-20.7299277273801,-19.6579889234461,
-6.84641998651614));
#74660=CARTESIAN_POINT('Ctrl Pts',(-20.7225805835101,-19.6781103655001,
-6.84500601987795));
#74661=CARTESIAN_POINT('Origin',(-18.734,-18.952,0.));
#74662=CARTESIAN_POINT('',(-20.7225805821268,-19.6781103692884,-6.04247206352563));
#74663=CARTESIAN_POINT('',(-20.722580459427,-19.6781107053232,-6.26710642520023));
#74664=CARTESIAN_POINT('',(-20.7225805821191,-19.6781103693095,0.));
#74665=CARTESIAN_POINT('Ctrl Pts',(-20.722580459427,-19.6781107053232,-6.26710642520023));
#74666=CARTESIAN_POINT('Ctrl Pts',(-20.7522829120589,-19.5967653726242,
-6.27277691375044));
#74667=CARTESIAN_POINT('Ctrl Pts',(-20.7769957147056,-19.5135926739805,
-6.27836345422882));
#74668=CARTESIAN_POINT('Ctrl Pts',(-20.8065479309516,-19.3858237632587,
-6.28658119025069));
#74669=CARTESIAN_POINT('Ctrl Pts',(-20.8151860571151,-19.3422858497125,
-6.28932042021308));
#74670=CARTESIAN_POINT('Ctrl Pts',(-20.8243855590297,-19.2868388869226,
-6.29273471116654));
#74671=CARTESIAN_POINT('Ctrl Pts',(-20.8262235216218,-19.2751557056022,
-6.29345001935078));
#74672=CARTESIAN_POINT('Ctrl Pts',(-20.829011487268,-19.2564119044014,-6.29459117866218));
#74673=CARTESIAN_POINT('Ctrl Pts',(-20.8300239038893,-19.2493609516757,
-6.29501899909521));
#74674=CARTESIAN_POINT('Ctrl Pts',(-20.8318772341774,-19.235973529657,-6.29582857368071));
#74675=CARTESIAN_POINT('Ctrl Pts',(-20.8327250735656,-19.2296381137333,
-6.2962105427308));
#74676=CARTESIAN_POINT('Ctrl Pts',(-20.8345859301686,-19.2152372049915,
-6.29707621867975));
#74677=CARTESIAN_POINT('Ctrl Pts',(-20.8355812164636,-19.2071694917844,
-6.29755936090405));
#74678=CARTESIAN_POINT('Ctrl Pts',(-20.8380346041774,-19.186293726902,-6.29880491120655));
#74679=CARTESIAN_POINT('Ctrl Pts',(-20.8394222482478,-19.173477614248,-6.29956509812174));
#74680=CARTESIAN_POINT('Ctrl Pts',(-20.8476032823545,-19.0908752941647,
-6.30443707438618));
#74681=CARTESIAN_POINT('Ctrl Pts',(-20.8510436183048,-19.0207966598717,
-6.30844173449181));
#74682=CARTESIAN_POINT('Ctrl Pts',(-20.8508787730343,-18.7582834169534,
-6.32314072120312));
#74683=CARTESIAN_POINT('Ctrl Pts',(-20.8245352117492,-18.5668343657836,
-6.33317505048021));
#74684=CARTESIAN_POINT('Ctrl Pts',(-20.7592947599496,-18.3336572753103,
-6.34683377332967));
#74685=CARTESIAN_POINT('Ctrl Pts',(-20.7441979055401,-18.2862146546721,
-6.34969727122593));
#74686=CARTESIAN_POINT('Ctrl Pts',(-20.7248154855874,-18.2319974235725,
-6.35311518075376));
#74687=CARTESIAN_POINT('Ctrl Pts',(-20.7221455095431,-18.224657277244,-6.35358104992598));
#74688=CARTESIAN_POINT('Ctrl Pts',(-20.7178168236286,-18.2129590312568,
-6.35432879726889));
#74689=CARTESIAN_POINT('Ctrl Pts',(-20.7161841985248,-18.2085912662877,
-6.35460916292821));
#74690=CARTESIAN_POINT('Ctrl Pts',(-20.71326896642,-18.2008700182166,-6.35510693818837));
#74691=CARTESIAN_POINT('Ctrl Pts',(-20.7119922425317,-18.197514361109,-6.35532399424251));
#74692=CARTESIAN_POINT('Ctrl Pts',(-20.7092701408979,-18.190414167292,-6.35578481427573));
#74693=CARTESIAN_POINT('Ctrl Pts',(-20.7078226713603,-18.1866705470788,
-6.3560286972433));
#74694=CARTESIAN_POINT('Ctrl Pts',(-20.7038921045113,-18.1765901617635,
-6.35668781580685));
#74695=CARTESIAN_POINT('Ctrl Pts',(-20.7013891054747,-18.1702612806059,
-6.35710422051401));
#74696=CARTESIAN_POINT('Ctrl Pts',(-20.6888792594576,-18.139070523753,-6.35916878035654));
#74697=CARTESIAN_POINT('Ctrl Pts',(-20.6784319312075,-18.1143893734034,
-6.36084140787467));
#74698=CARTESIAN_POINT('Ctrl Pts',(-20.6469617788922,-18.0438068633169,
-6.36572426776327));
#74699=CARTESIAN_POINT('Ctrl Pts',(-20.6247626639235,-17.9984521986412,
-6.36898510632641));
#74700=CARTESIAN_POINT('Ctrl Pts',(-20.5384183339973,-17.836937373781,-6.38094763674447));
#74701=CARTESIAN_POINT('Ctrl Pts',(-20.4650107302126,-17.72607384636,-6.3898158399104));
#74702=CARTESIAN_POINT('Ctrl Pts',(-20.3168837441426,-17.5424516024276,
-6.40514176592233));
#74703=CARTESIAN_POINT('Ctrl Pts',(-20.2462642351261,-17.4669377121572,
-6.41168271063618));
#74704=CARTESIAN_POINT('Ctrl Pts',(-20.1600892166794,-17.3873416507626,
-6.41884336375736));
#74705=CARTESIAN_POINT('Ctrl Pts',(-20.1496786628018,-17.37791609424,-6.41969617205793));
#74706=CARTESIAN_POINT('Ctrl Pts',(-20.1329049466645,-17.3630304525861,
-6.42105106458451));
#74707=CARTESIAN_POINT('Ctrl Pts',(-20.1266019391698,-17.3575034918229,
-6.42155594954601));
#74708=CARTESIAN_POINT('Ctrl Pts',(-20.1153950607495,-17.3477935835852,
-6.42244625021074));
#74709=CARTESIAN_POINT('Ctrl Pts',(-20.1105046349862,-17.3435953458113,
-6.42283229861664));
#74710=CARTESIAN_POINT('Ctrl Pts',(-20.100317802618,-17.3349308426697,-6.42363140074097));
#74711=CARTESIAN_POINT('Ctrl Pts',(-20.0950184851612,-17.3304681063441,
-6.4240443065721));
#74712=CARTESIAN_POINT('Ctrl Pts',(-20.0812910654333,-17.3190224817341,
-6.42510678284943));
#74713=CARTESIAN_POINT('Ctrl Pts',(-20.0728304798146,-17.3120787386936,
-6.42575475548946));
#74714=CARTESIAN_POINT('Ctrl Pts',(-20.0366931800307,-17.2828863273493,
-6.42849395872503));
#74715=CARTESIAN_POINT('Ctrl Pts',(-20.0085118961594,-17.2612695018461,
-6.43055985079432));
#74716=CARTESIAN_POINT('Ctrl Pts',(-19.9330683713103,-17.2063583904643,
-6.43592265549204));
#74717=CARTESIAN_POINT('Ctrl Pts',(-19.8849624544593,-17.1742723086868,
-6.43917563760426));
#74718=CARTESIAN_POINT('Ctrl Pts',(-19.6972068262767,-17.0598619808836,
-6.45137513556485));
#74719=CARTESIAN_POINT('Ctrl Pts',(-19.549598372377,-16.9917072816964,-6.45992615368772));
#74720=CARTESIAN_POINT('Ctrl Pts',(-19.3750799293361,-16.9342846186329,
-6.47018693705132));
#74721=CARTESIAN_POINT('Ctrl Pts',(-19.3543878741379,-16.9278266698602,
-6.47140655612698));
#74722=CARTESIAN_POINT('Ctrl Pts',(-19.2933234967709,-16.9097928647942,
-6.47502422703232));
#74723=CARTESIAN_POINT('Ctrl Pts',(-19.2527040405183,-16.8991000156803,
-6.4774541115432));
#74724=CARTESIAN_POINT('Ctrl Pts',(-19.2045513088841,-16.8879443372843,
-6.48039070956155));
#74725=CARTESIAN_POINT('Ctrl Pts',(-19.1972972546151,-16.8863040002784,
-6.48083458362917));
#74726=CARTESIAN_POINT('Ctrl Pts',(-19.1855410114021,-16.8837106362707,
-6.481556568));
#74727=CARTESIAN_POINT('Ctrl Pts',(-19.1810440223166,-16.8827339904478,
-6.48183336043624));
#74728=CARTESIAN_POINT('Ctrl Pts',(-19.173048981748,-16.8810249242269,-6.48232661751927));
#74729=CARTESIAN_POINT('Ctrl Pts',(-19.16955222348,-16.8802866913469,-6.48254274612517));
#74730=CARTESIAN_POINT('Ctrl Pts',(-19.1620433867143,-16.8787212827171,
-6.48300771786059));
#74731=CARTESIAN_POINT('Ctrl Pts',(-19.1580308316259,-16.8778969086322,
-6.48325671146392));
#74732=CARTESIAN_POINT('Ctrl Pts',(-19.1469794989126,-16.8756598366607,
-6.48394387745948));
#74733=CARTESIAN_POINT('Ctrl Pts',(-19.1399359648255,-16.8742713051324,
-6.48438339157216));
#74734=CARTESIAN_POINT('Ctrl Pts',(-19.10181476387,-16.866957498513,-6.48677001261174));
#74735=CARTESIAN_POINT('Ctrl Pts',(-19.0706160601182,-16.8616939666992,
-6.48875145077311));
#74736=CARTESIAN_POINT('Ctrl Pts',(-18.8775506369572,-16.8335559602815,
-6.50113860295273));
#74737=CARTESIAN_POINT('Ctrl Pts',(-18.7136066526049,-16.8287958513289,
-6.51214893227153));
#74738=CARTESIAN_POINT('Ctrl Pts',(-18.4341379738477,-16.8530782226375,
-6.53047402769161));
#74739=CARTESIAN_POINT('Ctrl Pts',(-18.3185533953526,-16.8728651239564,
-6.53793080217616));
#74740=CARTESIAN_POINT('Ctrl Pts',(-18.1913415586007,-16.9056825537609,
-6.54595268826156));
#74741=CARTESIAN_POINT('Ctrl Pts',(-18.1775384319861,-16.9093928880337,
-6.54682085688366));
#74742=CARTESIAN_POINT('Ctrl Pts',(-18.1556307548697,-16.9155203142669,
-6.54819541176844));
#74743=CARTESIAN_POINT('Ctrl Pts',(-18.1475014691584,-16.9178466206608,
-6.54870472773245));
#74744=CARTESIAN_POINT('Ctrl Pts',(-18.1331893056846,-16.9220351725402,
-6.54960017024048));
#74745=CARTESIAN_POINT('Ctrl Pts',(-18.1270006426208,-16.9238771061146,
-6.54998695320867));
#74746=CARTESIAN_POINT('Ctrl Pts',(-18.1142184373658,-16.927745225341,-6.55078500960992));
#74747=CARTESIAN_POINT('Ctrl Pts',(-18.1076261696227,-16.9297753822928,
-6.55119614781788));
#74748=CARTESIAN_POINT('Ctrl Pts',(-18.0907312520088,-16.9350688885102,
-6.55224873715808));
#74749=CARTESIAN_POINT('Ctrl Pts',(-18.0804433745375,-16.9383789992883,
-6.55288864768084));
#74750=CARTESIAN_POINT('Ctrl Pts',(-18.0376200282087,-16.9525201241054,
-6.55554835816367));
#74751=CARTESIAN_POINT('Ctrl Pts',(-18.0053237106633,-16.9640624001404,
-6.55754465093477));
#74752=CARTESIAN_POINT('Ctrl Pts',(-17.9219260024534,-16.9961733659085,
-6.56268609096014));
#74753=CARTESIAN_POINT('Ctrl Pts',(-17.8713207952001,-17.017960901597,-6.56579190216776));
#74754=CARTESIAN_POINT('Ctrl Pts',(-17.7229741070182,-17.0888128347816,
-6.57493326333654));
#74755=CARTESIAN_POINT('Ctrl Pts',(-17.6281231247613,-17.1434986888472,
-6.5808200738016));
#74756=CARTESIAN_POINT('Ctrl Pts',(-17.5024553388562,-17.2295499260154,
-6.58911213608491));
#74757=CARTESIAN_POINT('Ctrl Pts',(-17.4677390864689,-17.2549084825652,
-6.59146172692335));
#74758=CARTESIAN_POINT('Ctrl Pts',(-17.3741943210367,-17.3277075793914,
-6.59802361195137));
#74759=CARTESIAN_POINT('Ctrl Pts',(-17.3171021846353,-17.3772633997974,
-6.60229272212173));
#74760=CARTESIAN_POINT('Ctrl Pts',(-17.2559606255376,-17.4363553393903,
-6.60733217674834));
#74761=CARTESIAN_POINT('Ctrl Pts',(-17.2491787461259,-17.4429986858368,
-6.60789806543709));
#74762=CARTESIAN_POINT('Ctrl Pts',(-17.2391916072032,-17.4529143295949,
-6.60874213335978));
#74763=CARTESIAN_POINT('Ctrl Pts',(-17.2359518077676,-17.4561518822973,
-6.6090176424153));
#74764=CARTESIAN_POINT('Ctrl Pts',(-17.2302042609199,-17.4619328428253,
-6.60950949241245));
#74765=CARTESIAN_POINT('Ctrl Pts',(-17.227692418761,-17.4644721084171,-6.60972550458597));
#74766=CARTESIAN_POINT('Ctrl Pts',(-17.2223036025189,-17.4699474035801,
-6.61019123021394));
#74767=CARTESIAN_POINT('Ctrl Pts',(-17.2194287921008,-17.4728854161186,
-6.61044109942881));
#74768=CARTESIAN_POINT('Ctrl Pts',(-17.211511719523,-17.481023825935,-6.61113309750282));
#74769=CARTESIAN_POINT('Ctrl Pts',(-17.2064876187868,-17.4862417011649,
-6.61157659884844));
#74770=CARTESIAN_POINT('Ctrl Pts',(-17.1790233510643,-17.5150597938577,
-6.6140245931114));
#74771=CARTESIAN_POINT('Ctrl Pts',(-17.1571045790015,-17.5391482398456,
-6.61606549334081));
#74772=CARTESIAN_POINT('Ctrl Pts',(-17.029071351026,-17.686546842809,-6.62847213283241));
#74773=CARTESIAN_POINT('Ctrl Pts',(-16.9369055296477,-17.821245919886,-6.63942730611795));
#74774=CARTESIAN_POINT('Ctrl Pts',(-16.8066268614934,-18.0685044158201,
-6.65768272269842));
#74775=CARTESIAN_POINT('Ctrl Pts',(-16.7608186248174,-18.1761812535905,
-6.66512290945199));
#74776=CARTESIAN_POINT('Ctrl Pts',(-16.7196357938293,-18.3006705698452,
-6.67312935843537));
#74777=CARTESIAN_POINT('Ctrl Pts',(-16.7152852999757,-18.314282070732,-6.67399732649369));
#74778=CARTESIAN_POINT('Ctrl Pts',(-16.7085806033823,-18.3360156284829,
-6.67537162484848));
#74779=CARTESIAN_POINT('Ctrl Pts',(-16.7061367276736,-18.344109360051,-6.67588088314543));
#74780=CARTESIAN_POINT('Ctrl Pts',(-16.7019120785144,-18.3584097638266,
-6.67677625857528));
#74781=CARTESIAN_POINT('Ctrl Pts',(-16.7001111039519,-18.364610309,-6.67716303182294));
#74782=CARTESIAN_POINT('Ctrl Pts',(-16.6964447786512,-18.3774520878494,
-6.67796110101941));
#74783=CARTESIAN_POINT('Ctrl Pts',(-16.6945834619512,-18.3840944009193,
-6.67837226158113));
#74784=CARTESIAN_POINT('Ctrl Pts',(-16.6898890442752,-18.4011676942213,
-6.67942497614906));
#74785=CARTESIAN_POINT('Ctrl Pts',(-16.6871032805823,-18.4116115702577,
-6.68006498882599));
#74786=CARTESIAN_POINT('Ctrl Pts',(-16.6758102423518,-18.4552900204834,
-6.68272569202054));
#74787=CARTESIAN_POINT('Ctrl Pts',(-16.6680311666412,-18.4887086678556,
-6.68472285294477));
#74788=CARTESIAN_POINT('Ctrl Pts',(-16.6498822315711,-18.5762622847695,
-6.68986703424781));
#74789=CARTESIAN_POINT('Ctrl Pts',(-16.6408076643616,-18.6306400852839,
-6.69297466354843));
#74790=CARTESIAN_POINT('Ctrl Pts',(-16.6200900399427,-18.7937895408449,
-6.70211919669863));
#74791=CARTESIAN_POINT('Ctrl Pts',(-16.6147400615673,-18.9031731072094,
-6.70800737156691));
#74792=CARTESIAN_POINT('Ctrl Pts',(-16.6191735951262,-19.0582981501148,
-6.71645648286419));
#74793=CARTESIAN_POINT('Ctrl Pts',(-16.6219707858252,-19.1040604441326,
-6.71896277593144));
#74794=CARTESIAN_POINT('Ctrl Pts',(-16.6283556179594,-19.1721332981296,
-6.72275427608508));
#74795=CARTESIAN_POINT('Ctrl Pts',(-16.6308183899938,-19.1945365906223,
-6.72401242111201));
#74796=CARTESIAN_POINT('Ctrl Pts',(-16.6344001338201,-19.2229362854735,
-6.72562505655993));
#74797=CARTESIAN_POINT('Ctrl Pts',(-16.6351880138896,-19.2289734908284,
-6.72596889247919));
#74798=CARTESIAN_POINT('Ctrl Pts',(-16.6421026002959,-19.2802329316424,
-6.72889756666278));
#74799=CARTESIAN_POINT('Ctrl Pts',(-16.6496635822766,-19.3252460583367,
-6.73153084884893));
#74800=CARTESIAN_POINT('Ctrl Pts',(-16.6601768009813,-19.3774461257432,
-6.73469309994365));
#74801=CARTESIAN_POINT('Ctrl Pts',(-16.6617216040197,-19.384907972089,-6.73514774646076));
#74802=CARTESIAN_POINT('Ctrl Pts',(-16.6642649460114,-19.3968674306772,
-6.73588086185389));
#74803=CARTESIAN_POINT('Ctrl Pts',(-16.6652379567274,-19.4013704841021,
-6.73615790999352));
#74804=CARTESIAN_POINT('Ctrl Pts',(-16.6669938388295,-19.409370056143,-6.73665193556535));
#74805=CARTESIAN_POINT('Ctrl Pts',(-16.6677708968192,-19.4128678026972,
-6.73686857783967));
#74806=CARTESIAN_POINT('Ctrl Pts',(-16.6694442848269,-19.4203108661067,
-6.73733095349621));
#74807=CARTESIAN_POINT('Ctrl Pts',(-16.67034303185,-19.4242555299196,-6.7375768182143));
#74808=CARTESIAN_POINT('Ctrl Pts',(-16.6728164511585,-19.4349696506205,
-6.73824678468645));
#74809=CARTESIAN_POINT('Ctrl Pts',(-16.6744131455428,-19.4417338984473,
-6.73867212111415));
#74810=CARTESIAN_POINT('Ctrl Pts',(-16.6827429505346,-19.4762610347788,
-6.74085483072734));
#74811=CARTESIAN_POINT('Ctrl Pts',(-16.690003879291,-19.5038920072432,-6.74264009147455));
#74812=CARTESIAN_POINT('Ctrl Pts',(-16.7130202464255,-19.5847829142683,
-6.74796360774868));
#74813=CARTESIAN_POINT('Ctrl Pts',(-16.7303144179089,-19.6375775834551,
-6.75156300851509));
#74814=CARTESIAN_POINT('Ctrl Pts',(-16.7982331468631,-19.8202899871938,
-6.76433115205645));
#74815=CARTESIAN_POINT('Ctrl Pts',(-16.8595957319666,-19.9458482870958,
-6.77364484468825));
#74816=CARTESIAN_POINT('Ctrl Pts',(-16.9801585301175,-20.1410464608048,
-6.78845579730063));
#74817=CARTESIAN_POINT('Ctrl Pts',(-17.0323003627838,-20.2145424454453,
-6.79412862371263));
#74818=CARTESIAN_POINT('Ctrl Pts',(-17.0976038733076,-20.2951622599452,
-6.80045885254198));
#74819=CARTESIAN_POINT('Ctrl Pts',(-17.1063409359772,-20.3057367266937,
-6.80129157022892));
#74820=CARTESIAN_POINT('Ctrl Pts',(-17.1205207373237,-20.3225627848582,
-6.80262069699413));
#74821=CARTESIAN_POINT('Ctrl Pts',(-17.1258983778,-20.3288684955553,-6.80311974208911));
#74822=CARTESIAN_POINT('Ctrl Pts',(-17.1355143198483,-20.3400107641331,
-6.80400330668057));
#74823=CARTESIAN_POINT('Ctrl Pts',(-17.1397378667413,-20.3448598647644,
-6.80438842776142));
#74824=CARTESIAN_POINT('Ctrl Pts',(-17.1485857338772,-20.3549252283744,
-6.80518911371549));
#74825=CARTESIAN_POINT('Ctrl Pts',(-17.1532138612621,-20.3601380532445,
-6.80560451329396));
#74826=CARTESIAN_POINT('Ctrl Pts',(-17.1653039699175,-20.3736208479004,
-6.80668089360052));
#74827=CARTESIAN_POINT('Ctrl Pts',(-17.1728056838422,-20.3818550221435,
-6.80734019483284));
#74828=CARTESIAN_POINT('Ctrl Pts',(-17.2057051598498,-20.4173991707385,
-6.81019518318211));
#74829=CARTESIAN_POINT('Ctrl Pts',(-17.2317580123588,-20.4440955428683,
-6.81236272837021));
#74830=CARTESIAN_POINT('Ctrl Pts',(-17.3028866992972,-20.5132284937725,
-6.81805484253141));
#74831=CARTESIAN_POINT('Ctrl Pts',(-17.3491420227038,-20.5544009904482,
-6.82152807009403));
#74832=CARTESIAN_POINT('Ctrl Pts',(-17.5072090051151,-20.6831338878177,
-6.83280485535002));
#74833=CARTESIAN_POINT('Ctrl Pts',(-17.6260116162018,-20.7614750704277,
-6.84034767604244));
#74834=CARTESIAN_POINT('Ctrl Pts',(-17.8186314866175,-20.8623635136665,
-6.85238551067464));
#74835=CARTESIAN_POINT('Ctrl Pts',(-17.8873256450474,-20.8937848073749,
-6.85665147002291));
#74836=CARTESIAN_POINT('Ctrl Pts',(-17.9663619226266,-20.9249446671622,
-6.86168670128342));
#74837=CARTESIAN_POINT('Ctrl Pts',(-17.9752046884064,-20.9283624528559,
-6.8622518079189));
#74838=CARTESIAN_POINT('Ctrl Pts',(-17.9883506908276,-20.9333422375274,
-6.86309493026967));
#74839=CARTESIAN_POINT('Ctrl Pts',(-17.9926366590347,-20.9349499111801,
-6.86337028448628));
#74840=CARTESIAN_POINT('Ctrl Pts',(-18.0002758518047,-20.9377871563594,
-6.86386196523651));
#74841=CARTESIAN_POINT('Ctrl Pts',(-18.0036270065953,-20.9390221554576,
-6.86407796387979));
#74842=CARTESIAN_POINT('Ctrl Pts',(-18.0108435161693,-20.9416609286274,
-6.86454378281918));
#74843=CARTESIAN_POINT('Ctrl Pts',(-18.0147097841405,-20.9430619015281,
-6.86479375952265));
#74844=CARTESIAN_POINT('Ctrl Pts',(-18.0254049015843,-20.9469021454816,
-6.86548635139786));
#74845=CARTESIAN_POINT('Ctrl Pts',(-18.0322421646884,-20.9493175813126,
-6.86593034285788));
#74846=CARTESIAN_POINT('Ctrl Pts',(-18.0699627717014,-20.9624257455144,
-6.86838601277451));
#74847=CARTESIAN_POINT('Ctrl Pts',(-18.1010763267448,-20.9724367028159,
-6.8704343626453));
#74848=CARTESIAN_POINT('Ctrl Pts',(-18.2882853699942,-21.0279239049622,
-6.88284352534821));
#74849=CARTESIAN_POINT('Ctrl Pts',(-18.44896241195,-21.0560140477838,-6.89379189706699));
#74850=CARTESIAN_POINT('Ctrl Pts',(-18.7278429650211,-21.0722090017009,
-6.91203860527139));
#74851=CARTESIAN_POINT('Ctrl Pts',(-18.8447906932749,-21.0693231544684,
-6.91947663997359));
#74852=CARTESIAN_POINT('Ctrl Pts',(-18.9751271092756,-21.0552714723962,
-6.92748108555126));
#74853=CARTESIAN_POINT('Ctrl Pts',(-18.9893179661189,-21.0535960414207,
-6.9283490271902));
#74854=CARTESIAN_POINT('Ctrl Pts',(-19.0118766208041,-21.0507008027958,
-6.92972329175296));
#74855=CARTESIAN_POINT('Ctrl Pts',(-19.0202557616169,-21.0495743415254,
-6.93023254245332));
#74856=CARTESIAN_POINT('Ctrl Pts',(-19.0350218816356,-21.0474991089574,
-6.93112790904712));
#74857=CARTESIAN_POINT('Ctrl Pts',(-19.0414116473184,-21.0465712614734,
-6.93151468101459));
#74858=CARTESIAN_POINT('Ctrl Pts',(-19.0546190451169,-21.0445916973954,
-6.93231275189821));
#74859=CARTESIAN_POINT('Ctrl Pts',(-19.0614359894512,-21.04353586119,-6.93272391540586));
#74860=CARTESIAN_POINT('Ctrl Pts',(-19.078921087689,-21.0407401170678,-6.93377664647683));
#74861=CARTESIAN_POINT('Ctrl Pts',(-19.0895813806296,-21.038951777519,-6.93441667261602));
#74862=CARTESIAN_POINT('Ctrl Pts',(-19.1340181229977,-21.0311468252706,
-6.93707750666116));
#74863=CARTESIAN_POINT('Ctrl Pts',(-19.1676606140742,-21.0243910558106,
-6.93907478201967));
#74864=CARTESIAN_POINT('Ctrl Pts',(-19.2548778709147,-21.0046598440315,
-6.94421932469722));
#74865=CARTESIAN_POINT('Ctrl Pts',(-19.3081373223509,-20.9904045654281,
-6.94732719367996));
#74866=CARTESIAN_POINT('Ctrl Pts',(-19.4635933629355,-20.9422181057136,
-6.95637679664332));
#74867=CARTESIAN_POINT('Ctrl Pts',(-19.5638266130352,-20.9025546091438,
-6.96217621955508));
#74868=CARTESIAN_POINT('Ctrl Pts',(-19.7686877885259,-20.8028267082135,
-6.97457694609246));
#74869=CARTESIAN_POINT('Ctrl Pts',(-19.8720744085514,-20.7411105447019,
-6.98117295068701));
#74870=CARTESIAN_POINT('Ctrl Pts',(-19.9773653041375,-20.6654240535901,
-6.98885801498727));
#74871=CARTESIAN_POINT('Ctrl Pts',(-19.985042292683,-20.6598268182876,-6.98942432887112));
#74872=CARTESIAN_POINT('Ctrl Pts',(-19.9963650565162,-20.6514541639817,
-6.99026891085024));
#74873=CARTESIAN_POINT('Ctrl Pts',(-20.0000400377689,-20.6487181891077,
-6.99054450404216));
#74874=CARTESIAN_POINT('Ctrl Pts',(-20.0064391953981,-20.643921736002,-6.99102701716286));
#74875=CARTESIAN_POINT('Ctrl Pts',(-20.0091673014988,-20.6418665686252,
-6.99123356436192));
#74876=CARTESIAN_POINT('Ctrl Pts',(-20.0150562182121,-20.6374078832479,
-6.99168125696093));
#74877=CARTESIAN_POINT('Ctrl Pts',(-20.0182151964123,-20.6350021080908,
-6.9919225576278));
#74878=CARTESIAN_POINT('Ctrl Pts',(-20.0266049605384,-20.6285753623349,
-6.99256642937428));
#74879=CARTESIAN_POINT('Ctrl Pts',(-20.0318236998357,-20.6245388399348,
-6.99297007424193));
#74880=CARTESIAN_POINT('Ctrl Pts',(-20.0434209072886,-20.6154818237276,
-6.99387391430647));
#74881=CARTESIAN_POINT('Ctrl Pts',(-20.0497895078531,-20.6104489309782,
-6.99437492431482));
#74882=CARTESIAN_POINT('Ctrl Pts',(-20.0690124349333,-20.5950772723018,
-6.99590097655186));
#74883=CARTESIAN_POINT('Ctrl Pts',(-20.0817747057316,-20.5846250124554,
-6.99693302824633));
#74884=CARTESIAN_POINT('Ctrl Pts',(-20.1289520063921,-20.5450568080324,
-7.00081521503053));
#74885=CARTESIAN_POINT('Ctrl Pts',(-20.1625547210036,-20.5149945565157,
-7.00371569066448));
#74886=CARTESIAN_POINT('Ctrl Pts',(-20.2500895844626,-20.4315004725714,
-7.01158889597075));
#74887=CARTESIAN_POINT('Ctrl Pts',(-20.3021508636173,-20.3762020752341,
-7.01661527365881));
#74888=CARTESIAN_POINT('Ctrl Pts',(-20.4510455466623,-20.199963809805,-7.03185549933659));
#74889=CARTESIAN_POINT('Ctrl Pts',(-20.5377040853262,-20.0710742049076,
-7.0419423529683));
#74890=CARTESIAN_POINT('Ctrl Pts',(-20.6206410394289,-19.9126497532631,
-7.0529593810999));
#74891=CARTESIAN_POINT('Ctrl Pts',(-20.6313863131782,-19.8912484296231,
-7.05442203207489));
#74892=CARTESIAN_POINT('Ctrl Pts',(-20.6459733677997,-19.8609230029996,
-7.05645965424622));
#74893=CARTESIAN_POINT('Ctrl Pts',(-20.6501200623779,-19.8521483744456,
-7.0570451925395));
#74894=CARTESIAN_POINT('Ctrl Pts',(-20.6567308342652,-19.8379069304022,
-7.05798909874007));
#74895=CARTESIAN_POINT('Ctrl Pts',(-20.6592322466665,-19.8324576922908,
-7.05834875421579));
#74896=CARTESIAN_POINT('Ctrl Pts',(-20.6643974319548,-19.8210782565451,
-7.05909669053979));
#74897=CARTESIAN_POINT('Ctrl Pts',(-20.6670571110406,-19.8151462611903,
-7.05948482743104));
#74898=CARTESIAN_POINT('Ctrl Pts',(-20.6732798529584,-19.8010943865385,
-7.06040016366369));
#74899=CARTESIAN_POINT('Ctrl Pts',(-20.6768193260813,-19.7929641461986,
-7.06092655095774));
#74900=CARTESIAN_POINT('Ctrl Pts',(-20.6883950565319,-19.7659112964969,
-7.06266762262549));
#74901=CARTESIAN_POINT('Ctrl Pts',(-20.6962069166949,-19.7468935120836,
-7.06387468139385));
#74902=CARTESIAN_POINT('Ctrl Pts',(-20.7102289848657,-19.7112901289879,
-7.06610478058572));
#74903=CARTESIAN_POINT('Ctrl Pts',(-20.7165093627717,-19.6947374676077,
-7.06712985185229));
#74904=CARTESIAN_POINT('Ctrl Pts',(-20.7225805740154,-19.678110391503,-7.06814851970791));
#74905=CARTESIAN_POINT('Ctrl Pts',(-20.7225805835101,-19.6781103655001,
-6.84500601987795));
#74906=CARTESIAN_POINT('Ctrl Pts',(-20.7143219854172,-19.7007279847972,
-6.84341664278283));
#74907=CARTESIAN_POINT('Ctrl Pts',(-20.7056776273264,-19.7232044037876,
-6.84182487853371));
#74908=CARTESIAN_POINT('Ctrl Pts',(-20.6822899566468,-19.7810495426352,
-6.83770203086913));
#74909=CARTESIAN_POINT('Ctrl Pts',(-20.6669669703437,-19.8161734031987,
-6.83517286881883));
#74910=CARTESIAN_POINT('Ctrl Pts',(-20.6103476751077,-19.9369061608838,
-6.82641399128989));
#74911=CARTESIAN_POINT('Ctrl Pts',(-20.5642445701084,-20.0201428700487,
-6.82026486865833));
#74912=CARTESIAN_POINT('Ctrl Pts',(-20.4876288281751,-20.1388496640421,
-6.81139907214313));
#74913=CARTESIAN_POINT('Ctrl Pts',(-20.4612923602198,-20.176862367634,-6.80854270242055));
#74914=CARTESIAN_POINT('Ctrl Pts',(-20.4265842288022,-20.2236097438781,
-6.80500499427594));
#74915=CARTESIAN_POINT('Ctrl Pts',(-20.4193562061972,-20.2331741410964,
-6.80427979467784));
#74916=CARTESIAN_POINT('Ctrl Pts',(-20.4076825967969,-20.2483513473345,
-6.80312662672716));
#74917=CARTESIAN_POINT('Ctrl Pts',(-20.4032891848287,-20.2540037902906,
-6.80269661531298));
#74918=CARTESIAN_POINT('Ctrl Pts',(-20.3949230715704,-20.2646554468028,
-6.8018852212007));
#74919=CARTESIAN_POINT('Ctrl Pts',(-20.3909562691669,-20.269659172603,-6.80150361041117));
#74920=CARTESIAN_POINT('Ctrl Pts',(-20.3819261606153,-20.2809444918424,
-6.80064186669378));
#74921=CARTESIAN_POINT('Ctrl Pts',(-20.3768494431342,-20.2872152647369,
-6.80016227846972));
#74922=CARTESIAN_POINT('Ctrl Pts',(-20.3617613838255,-20.3056357385139,
-6.79875112185494));
#74923=CARTESIAN_POINT('Ctrl Pts',(-20.3516500886938,-20.3177031323707,
-6.79782360748397));
#74924=CARTESIAN_POINT('Ctrl Pts',(-20.2603445454015,-20.4242354505289,
-6.78960465912225));
#74925=CARTESIAN_POINT('Ctrl Pts',(-20.1710907798022,-20.5114810019239,
-6.78267611821987));
#74926=CARTESIAN_POINT('Ctrl Pts',(-19.9449935097697,-20.696494222655,-6.76672054894049));
#74927=CARTESIAN_POINT('Ctrl Pts',(-19.8031955937225,-20.786821706128,-6.75786063141456));
#74928=CARTESIAN_POINT('Ctrl Pts',(-19.6328541194331,-20.8688239755822,
-6.74686258294512));
#74929=CARTESIAN_POINT('Ctrl Pts',(-19.6133072136024,-20.8778690569118,
-6.74559506334164));
#74930=CARTESIAN_POINT('Ctrl Pts',(-19.5878766232969,-20.8891688883436,
-6.74393470548453));
#74931=CARTESIAN_POINT('Ctrl Pts',(-19.582115381972,-20.8916981431034,-6.74355781304137));
#74932=CARTESIAN_POINT('Ctrl Pts',(-19.5732577041436,-20.895539764418,-6.7429770922349));
#74933=CARTESIAN_POINT('Ctrl Pts',(-19.5701692144989,-20.8968705237624,
-6.74277437202766));
#74934=CARTESIAN_POINT('Ctrl Pts',(-19.5637954373323,-20.8995988495023,
-6.74235550462217));
#74935=CARTESIAN_POINT('Ctrl Pts',(-19.5605098099,-20.900995454047,-6.74213929977439));
#74936=CARTESIAN_POINT('Ctrl Pts',(-19.5530170090569,-20.9041580258165,
-6.74164561503926));
#74937=CARTESIAN_POINT('Ctrl Pts',(-19.5488076657731,-20.9059186998903,
-6.74136781969645));
#74938=CARTESIAN_POINT('Ctrl Pts',(-19.5378417976435,-20.9104638798799,
-6.74064301992948));
#74939=CARTESIAN_POINT('Ctrl Pts',(-19.5310765541438,-20.9132270056576,
-6.7401947735487));
#74940=CARTESIAN_POINT('Ctrl Pts',(-19.4877712048934,-20.9306531170134,
-6.7373191550399));
#74941=CARTESIAN_POINT('Ctrl Pts',(-19.4508448173797,-20.9443283463676,
-6.73483853185894));
#74942=CARTESIAN_POINT('Ctrl Pts',(-19.2327777342574,-21.0182398563808,
-6.72011012947499));
#74943=CARTESIAN_POINT('Ctrl Pts',(-19.0445337523876,-21.054785395015,-6.70717973171493));
#74944=CARTESIAN_POINT('Ctrl Pts',(-18.7989193959445,-21.0687214835421,
-6.69136696687255));
#74945=CARTESIAN_POINT('Ctrl Pts',(-18.7438094961671,-21.0696942558855,
-6.68787822026557));
#74946=CARTESIAN_POINT('Ctrl Pts',(-18.6544278808095,-21.0677820774067,
-6.682321199515));
#74947=CARTESIAN_POINT('Ctrl Pts',(-18.6201567100273,-21.066215089064,-6.6802144960893));
#74948=CARTESIAN_POINT('Ctrl Pts',(-18.57515544615,-21.0630599762427,-6.67747814418383));
#74949=CARTESIAN_POINT('Ctrl Pts',(-18.5643795816716,-21.0622214898092,
-6.67682515815192));
#74950=CARTESIAN_POINT('Ctrl Pts',(-18.5467375972623,-21.0607127291629,
-6.67575968085642));
#74951=CARTESIAN_POINT('Ctrl Pts',(-18.5398675938761,-21.0600913624076,
-6.67534566027352));
#74952=CARTESIAN_POINT('Ctrl Pts',(-18.5265730905179,-21.0588233829699,
-6.6745461476453));
#74953=CARTESIAN_POINT('Ctrl Pts',(-18.5201482788146,-21.0581809353846,
-6.67416052928455));
#74954=CARTESIAN_POINT('Ctrl Pts',(-18.5053175481295,-21.0566293782444,
-6.67327209800026));
#74955=CARTESIAN_POINT('Ctrl Pts',(-18.4969138991525,-21.0556992816254,
-6.67276995119458));
#74956=CARTESIAN_POINT('Ctrl Pts',(-18.4743220287201,-21.0530617707871,
-6.67142329969202));
#74957=CARTESIAN_POINT('Ctrl Pts',(-18.4601449959225,-21.0512609806989,
-6.67058173668987));
#74958=CARTESIAN_POINT('Ctrl Pts',(-18.3301963150198,-21.0334158426373,
-6.6628974703257));
#74959=CARTESIAN_POINT('Ctrl Pts',(-18.2159141693931,-21.0079527390782,
-6.65637169077549));
#74960=CARTESIAN_POINT('Ctrl Pts',(-17.9487676730689,-20.9247238206964,
-6.64105377620314));
#74961=CARTESIAN_POINT('Ctrl Pts',(-17.799362609964,-20.8584810782739,-6.63244520774425));
#74962=CARTESIAN_POINT('Ctrl Pts',(-17.6312115529206,-20.7593712013123,
-6.62123549888504));
#74963=CARTESIAN_POINT('Ctrl Pts',(-17.6037566214886,-20.7423303233863,
-6.61935066406941));
#74964=CARTESIAN_POINT('Ctrl Pts',(-17.5706533514501,-20.7207186864475,
-6.61699673764266));
#74965=CARTESIAN_POINT('Ctrl Pts',(-17.5646229467832,-20.7167375216916,
-6.61656454944253));
#74966=CARTESIAN_POINT('Ctrl Pts',(-17.5551975453834,-20.7104455175486,
-6.61588354107986));
#74967=CARTESIAN_POINT('Ctrl Pts',(-17.5517886243604,-20.7081554964885,
-6.61563610011723));
#74968=CARTESIAN_POINT('Ctrl Pts',(-17.5454268423729,-20.703854905758,-6.61517214672524));
#74969=CARTESIAN_POINT('Ctrl Pts',(-17.5424723998708,-20.7018467759582,
-6.61495579855911));
#74970=CARTESIAN_POINT('Ctrl Pts',(-17.5357367750153,-20.6972436148394,
-6.61446054399009));
#74971=CARTESIAN_POINT('Ctrl Pts',(-17.5319589462618,-20.694643777627,-6.61418131417358));
#74972=CARTESIAN_POINT('Ctrl Pts',(-17.520362212717,-20.6866074519778,-6.61331975655933));
#74973=CARTESIAN_POINT('Ctrl Pts',(-17.5125716462733,-20.6811305503357,
-6.61273477479369));
#74974=CARTESIAN_POINT('Ctrl Pts',(-17.4083391333826,-20.6067974239799,
-6.60482735084867));
#74975=CARTESIAN_POINT('Ctrl Pts',(-17.317818016391,-20.5300219586709,-6.59703648355805));
#74976=CARTESIAN_POINT('Ctrl Pts',(-17.1570251419339,-20.36861511464,-6.58198658575987));
#74977=CARTESIAN_POINT('Ctrl Pts',(-17.0859583110822,-20.2852704691975,
-6.57475560850043));
#74978=CARTESIAN_POINT('Ctrl Pts',(-16.9892643541347,-20.1522580379777,
-6.56418578683252));
#74979=CARTESIAN_POINT('Ctrl Pts',(-16.9586308567259,-20.1064639693811,
-6.56069855252346));
#74980=CARTESIAN_POINT('Ctrl Pts',(-16.9118770017224,-20.0303007865398,
-6.55514365851298));
#74981=CARTESIAN_POINT('Ctrl Pts',(-16.8946498109096,-20.000644794519,-6.55303760619089));
#74982=CARTESIAN_POINT('Ctrl Pts',(-16.8729501547281,-19.9611081523475,
-6.55030196344546));
#74983=CARTESIAN_POINT('Ctrl Pts',(-16.8678230108253,-19.9515945385897,
-6.54964905059574));
#74984=CARTESIAN_POINT('Ctrl Pts',(-16.8595430786369,-19.935945032989,-6.54858366210338));
#74985=CARTESIAN_POINT('Ctrl Pts',(-16.8563470787238,-19.9298323409278,
-6.54816965763335));
#74986=CARTESIAN_POINT('Ctrl Pts',(-16.8502172749656,-19.9179675646923,
-6.54737015497548));
#74987=CARTESIAN_POINT('Ctrl Pts',(-16.8472798033342,-19.9122174712506,
-6.54698453058293));
#74988=CARTESIAN_POINT('Ctrl Pts',(-16.8405565056246,-19.898906662827,-6.54609605518229));
#74989=CARTESIAN_POINT('Ctrl Pts',(-16.8367895611247,-19.8913364936408,
-6.54559387050442));
#74990=CARTESIAN_POINT('Ctrl Pts',(-16.8267775234656,-19.8709100620896,
-6.54424705036412));
#74991=CARTESIAN_POINT('Ctrl Pts',(-16.8206170346202,-19.858012648875,-6.54340535776289));
#74992=CARTESIAN_POINT('Ctrl Pts',(-16.7652105321332,-19.7389291661411,
-6.53571092690519));
#74993=CARTESIAN_POINT('Ctrl Pts',(-16.7247165888992,-19.6288862082935,
-6.52917611752084));
#74994=CARTESIAN_POINT('Ctrl Pts',(-16.649971561305,-19.3584910897564,-6.51381941340986));
#74995=CARTESIAN_POINT('Ctrl Pts',(-16.6248187145037,-19.1964415528838,
-6.50518270586816));
#74996=CARTESIAN_POINT('Ctrl Pts',(-16.6173417152226,-19.0014918697698,
-6.49397028877299));
#74997=CARTESIAN_POINT('Ctrl Pts',(-16.6168382986956,-18.9698277186779,
-6.4921221548721));
#74998=CARTESIAN_POINT('Ctrl Pts',(-16.6170921265095,-18.9309851370272,
-6.48980907832235));
#74999=CARTESIAN_POINT('Ctrl Pts',(-16.6171755905183,-18.9238045150507,
-6.48937954428305));
#75000=CARTESIAN_POINT('Ctrl Pts',(-16.6173640441411,-18.9125283082934,
-6.48870179743376));
#75001=CARTESIAN_POINT('Ctrl Pts',(-16.6174443928772,-18.9084322896644,
-6.48845494207859));
#75002=CARTESIAN_POINT('Ctrl Pts',(-16.6176170939468,-18.9007636118522,
-6.48799147988173));
#75003=CARTESIAN_POINT('Ctrl Pts',(-16.6177066036871,-18.8971909445545,
-6.48777503361597));
#75004=CARTESIAN_POINT('Ctrl Pts',(-16.6179320477313,-18.8890191128216,
-6.48727875032715));
#75005=CARTESIAN_POINT('Ctrl Pts',(-16.6180739294109,-18.8844201683435,
-6.48699858470329));
#75006=CARTESIAN_POINT('Ctrl Pts',(-16.6184842939782,-18.8723911015177,
-6.48626357535467));
#75007=CARTESIAN_POINT('Ctrl Pts',(-16.6187769262391,-18.8649619414311,
-6.48580743280859));
#75008=CARTESIAN_POINT('Ctrl Pts',(-16.6209807527879,-18.8156226721339,
-6.48276412425206));
#75009=CARTESIAN_POINT('Ctrl Pts',(-16.624098162374,-18.7737787654935,-6.48011647832541));
#75010=CARTESIAN_POINT('Ctrl Pts',(-16.6300173621386,-18.7171130862076,
-6.47646446287558));
#75011=CARTESIAN_POINT('Ctrl Pts',(-16.6317375859846,-18.7021850144727,
-6.47549605174676));
#75012=CARTESIAN_POINT('Ctrl Pts',(-16.6545632958296,-18.5210798102523,
-6.46367979187551));
#75013=CARTESIAN_POINT('Ctrl Pts',(-16.6951610935069,-18.3579522419709,
-6.45240533508982));
#75014=CARTESIAN_POINT('Ctrl Pts',(-16.7753516803641,-18.1465060216482,
-6.43782943095842));
#75015=CARTESIAN_POINT('Ctrl Pts',(-16.7984018495846,-18.0925905720646,
-6.43410940993404));
#75016=CARTESIAN_POINT('Ctrl Pts',(-16.8391184726181,-18.0073310203449,
-6.42822885809885));
#75017=CARTESIAN_POINT('Ctrl Pts',(-16.8553960358253,-17.9753614400452,
-6.42602408576242));
#75018=CARTESIAN_POINT('Ctrl Pts',(-16.8777100589974,-17.9341604679788,
-6.42318121114312));
#75019=CARTESIAN_POINT('Ctrl Pts',(-16.8830163610748,-17.9245423446355,
-6.42251743923023));
#75020=CARTESIAN_POINT('Ctrl Pts',(-16.8917953916259,-17.9089183641132,
-6.42143887014229));
#75021=CARTESIAN_POINT('Ctrl Pts',(-16.8952231543605,-17.902887598033,-6.42102247051382));
#75022=CARTESIAN_POINT('Ctrl Pts',(-16.9018912720787,-17.8912888665283,
-6.42022143194358));
#75023=CARTESIAN_POINT('Ctrl Pts',(-16.9051275171653,-17.8857186381904,
-6.4198366505565));
#75024=CARTESIAN_POINT('Ctrl Pts',(-16.9126232268814,-17.8729515367666,
-6.4189544765716));
#75025=CARTESIAN_POINT('Ctrl Pts',(-16.916900028782,-17.865764927226,-6.41845771995237));
#75026=CARTESIAN_POINT('Ctrl Pts',(-16.9284367184189,-17.8466378375732,
-6.4171349960188));
#75027=CARTESIAN_POINT('Ctrl Pts',(-16.9357725122799,-17.8347434536846,
-6.41631180721062));
#75028=CARTESIAN_POINT('Ctrl Pts',(-16.9966445312147,-17.7381973484278,
-6.40962267679503));
#75029=CARTESIAN_POINT('Ctrl Pts',(-17.0560120669031,-17.6573644910778,
-6.40398437651985));
#75030=CARTESIAN_POINT('Ctrl Pts',(-17.2321291162792,-17.4501412498993,
-6.38899950788371));
#75031=CARTESIAN_POINT('Ctrl Pts',(-17.3588741841571,-17.3332927326408,
-6.37997057777922));
#75032=CARTESIAN_POINT('Ctrl Pts',(-17.5307433376399,-17.2097438452632,
-6.36791119503487));
#75033=CARTESIAN_POINT('Ctrl Pts',(-17.5638129195058,-17.18736268972,-6.36559564730284));
#75034=CARTESIAN_POINT('Ctrl Pts',(-17.6039789913882,-17.1618043060634,
-6.36276379572246));
#75035=CARTESIAN_POINT('Ctrl Pts',(-17.6104873602938,-17.1577125517882,
-6.36230433879136));
#75036=CARTESIAN_POINT('Ctrl Pts',(-17.6205918606746,-17.1514364722087,
-6.36158986450907));
#75037=CARTESIAN_POINT('Ctrl Pts',(-17.6241725376006,-17.1492272174991,
-6.36133645841383));
#75038=CARTESIAN_POINT('Ctrl Pts',(-17.630796648954,-17.1451673975155,-6.36086721270737));
#75039=CARTESIAN_POINT('Ctrl Pts',(-17.6338381772874,-17.1433138330682,
-6.36065157397906));
#75040=CARTESIAN_POINT('Ctrl Pts',(-17.6406887430015,-17.1391626429884,
-6.3601654805608));
#75041=CARTESIAN_POINT('Ctrl Pts',(-17.6445003276663,-17.1368693570971,
-6.35989474979174));
#75042=CARTESIAN_POINT('Ctrl Pts',(-17.6542707535155,-17.1310327247085,
-6.35920013124528));
#75043=CARTESIAN_POINT('Ctrl Pts',(-17.6602397710093,-17.127506637175,-6.35877516278824));
#75044=CARTESIAN_POINT('Ctrl Pts',(-17.6951944725997,-17.1070887330212,
-6.35628349365683));
#75045=CARTESIAN_POINT('Ctrl Pts',(-17.72455935678,-17.0908595423594,-6.3541781573002));
#75046=CARTESIAN_POINT('Ctrl Pts',(-17.7705072620938,-17.0668726314496,
-6.35087960364614));
#75047=CARTESIAN_POINT('Ctrl Pts',(-17.7868276594351,-17.0586199608626,
-6.34970715444302));
#75048=CARTESIAN_POINT('Ctrl Pts',(-17.8254388926516,-17.0397197126319,
-6.34693470648031));
#75049=CARTESIAN_POINT('Ctrl Pts',(-17.8478131141558,-17.029248866828,-6.34532920737995));
#75050=CARTESIAN_POINT('Ctrl Pts',(-17.9113756774904,-17.0008475428734,
-6.34078022524983));
#75051=CARTESIAN_POINT('Ctrl Pts',(-17.9529585126555,-16.9838331618609,
-6.33781851446724));
#75052=CARTESIAN_POINT('Ctrl Pts',(-18.0975170120735,-16.9299874800686,
-6.32762836554599));
#75053=CARTESIAN_POINT('Ctrl Pts',(-18.2027950636094,-16.8998133596006,
-6.32039833415335));
#75054=CARTESIAN_POINT('Ctrl Pts',(-18.3638784916733,-16.8668788601433,
-6.3098304989886));
#75055=CARTESIAN_POINT('Ctrl Pts',(-18.4182309964562,-16.8579582491381,
-6.30634429873058));
#75056=CARTESIAN_POINT('Ctrl Pts',(-18.5068944892584,-16.8469376717436,
-6.30079085898782));
#75057=CARTESIAN_POINT('Ctrl Pts',(-18.5410147577039,-16.8435358122439,
-6.29868525194005));
#75058=CARTESIAN_POINT('Ctrl Pts',(-18.5859799076044,-16.8401534562664,
-6.29595009418729));
#75059=CARTESIAN_POINT('Ctrl Pts',(-18.5967617762978,-16.8394253980584,
-6.29529723139733));
#75060=CARTESIAN_POINT('Ctrl Pts',(-18.6144340908385,-16.8383679201721,
-6.29423190364988));
#75061=CARTESIAN_POINT('Ctrl Pts',(-18.6213213104347,-16.8379895718846,
-6.29381791020152));
#75062=CARTESIAN_POINT('Ctrl Pts',(-18.6346591961947,-16.8373222238807,
-6.29301841436067));
#75063=CARTESIAN_POINT('Ctrl Pts',(-18.6411095689713,-16.8370290637074,
-6.29263278583931));
#75064=CARTESIAN_POINT('Ctrl Pts',(-18.6560100706432,-16.8364201568125,
-6.29174428024787));
#75065=CARTESIAN_POINT('Ctrl Pts',(-18.6644609879816,-16.836125516257,-6.29124206965336));
#75066=CARTESIAN_POINT('Ctrl Pts',(-18.6872016712451,-16.8354690559113,
-6.28989513410677));
#75067=CARTESIAN_POINT('Ctrl Pts',(-18.701493867076,-16.8352013116252,-6.2890533528143));
#75068=CARTESIAN_POINT('Ctrl Pts',(-18.8329520607706,-16.8340703657281,
-6.28135185329706));
#75069=CARTESIAN_POINT('Ctrl Pts',(-18.9500047419029,-16.8427905052208,
-6.27481076412205));
#75070=CARTESIAN_POINT('Ctrl Pts',(-19.2275946151357,-16.8868348352363,
-6.25942584745279));
#75071=CARTESIAN_POINT('Ctrl Pts',(-19.3858917478135,-16.931216092929,-6.25076843480755));
#75072=CARTESIAN_POINT('Ctrl Pts',(-19.5663314778003,-17.0052368748225,
-6.23955363471204));
#75073=CARTESIAN_POINT('Ctrl Pts',(-19.5949288075185,-17.0177136431849,
-6.23773211010064));
#75074=CARTESIAN_POINT('Ctrl Pts',(-19.6297250736602,-17.0338194334036,
-6.23544866828161));
#75075=CARTESIAN_POINT('Ctrl Pts',(-19.6361965328241,-17.0368547035552,
-6.23502109578778));
#75076=CARTESIAN_POINT('Ctrl Pts',(-19.6463460525425,-17.0416779317097,
-6.23434575973968));
#75077=CARTESIAN_POINT('Ctrl Pts',(-19.6500345842939,-17.0434439060081,
-6.23409933766474));
#75078=CARTESIAN_POINT('Ctrl Pts',(-19.6569379622463,-17.0467736883354,
-6.23363623519491));
#75079=CARTESIAN_POINT('Ctrl Pts',(-19.6601539720458,-17.0483349558805,
-6.23341971263518));
#75080=CARTESIAN_POINT('Ctrl Pts',(-19.6675103600951,-17.0519292950798,
-6.23292265129036));
#75081=CARTESIAN_POINT('Ctrl Pts',(-19.6716480462529,-17.0539677514517,
-6.23264177999507));
#75082=CARTESIAN_POINT('Ctrl Pts',(-19.6824717821642,-17.0593441612441,
-6.23190372259834));
#75083=CARTESIAN_POINT('Ctrl Pts',(-19.689146809453,-17.0627039898041,-6.23144522047047));
#75084=CARTESIAN_POINT('Ctrl Pts',(-19.7338275216001,-17.0854910179538,
-6.22835436897585));
#75085=CARTESIAN_POINT('Ctrl Pts',(-19.7712532163773,-17.1060270722113,
-6.22565942242448));
#75086=CARTESIAN_POINT('Ctrl Pts',(-19.8142369740676,-17.1313328240116,
-6.22246030372404));
#75087=CARTESIAN_POINT('Ctrl Pts',(-19.8204255531634,-17.1350188770393,
-6.22199712856155));
#75088=CARTESIAN_POINT('Ctrl Pts',(-19.9612667908131,-17.2198837866833,
-6.21139886678943));
#75089=CARTESIAN_POINT('Ctrl Pts',(-20.086479596813,-17.3157810033686,-6.20082561343532));
#75090=CARTESIAN_POINT('Ctrl Pts',(-20.2683631252552,-17.4903510055799,
-6.18444648527678));
#75091=CARTESIAN_POINT('Ctrl Pts',(-20.3323175773567,-17.5605715644623,
-6.17842085925353));
#75092=CARTESIAN_POINT('Ctrl Pts',(-20.4046232468636,-17.6515531901783,
-6.17128278093974));
#75093=CARTESIAN_POINT('Ctrl Pts',(-20.4176410439852,-17.6684514713499,
-6.16998273407402));
#75094=CARTESIAN_POINT('Ctrl Pts',(-20.4357852638612,-17.6927554238908,
-6.16814850795982));
#75095=CARTESIAN_POINT('Ctrl Pts',(-20.4411229328079,-17.7000010850858,
-6.16760607468737));
#75096=CARTESIAN_POINT('Ctrl Pts',(-20.4502504309153,-17.7125581794305,
-6.16667348775311));
#75097=CARTESIAN_POINT('Ctrl Pts',(-20.4540621747525,-17.7178534590016,
-6.1662824868314));
#75098=CARTESIAN_POINT('Ctrl Pts',(-20.4613129495777,-17.7280250909617,
-6.16553570874941));
#75099=CARTESIAN_POINT('Ctrl Pts',(-20.4647559574677,-17.7328985191761,
-6.16517978076402));
#75100=CARTESIAN_POINT('Ctrl Pts',(-20.4736538370317,-17.7456067535594,
-6.16425644286757));
#75101=CARTESIAN_POINT('Ctrl Pts',(-20.4790764376013,-17.7534640726189,
-6.16369026905189));
#75102=CARTESIAN_POINT('Ctrl Pts',(-20.4973780555938,-17.7803705543315,
-6.16176721165222));
#75103=CARTESIAN_POINT('Ctrl Pts',(-20.5100000731756,-17.7995931595424,
-6.16042002013654));
#75104=CARTESIAN_POINT('Ctrl Pts',(-20.6162011652518,-17.9672217366862,
-6.14888906976616));
#75105=CARTESIAN_POINT('Ctrl Pts',(-20.6913089535726,-18.1265196452655,
-6.13945581009008));
#75106=CARTESIAN_POINT('Ctrl Pts',(-20.7729860249327,-18.3759800718239,
-6.12517350255245));
#75107=CARTESIAN_POINT('Ctrl Pts',(-20.7949379617914,-18.4602731565903,
-6.12040915521734));
#75108=CARTESIAN_POINT('Ctrl Pts',(-20.818900132923,-18.5827961291658,-6.11328128615683));
#75109=CARTESIAN_POINT('Ctrl Pts',(-20.8251640469048,-18.6201075595146,
-6.11108389291071));
#75110=CARTESIAN_POINT('Ctrl Pts',(-20.8314778231644,-18.6650625199462,
-6.10838294459277));
#75111=CARTESIAN_POINT('Ctrl Pts',(-20.8324907021525,-18.6725664565944,
-6.10793032174421));
#75112=CARTESIAN_POINT('Ctrl Pts',(-20.8340004993208,-18.6842232368771,
-6.10722422659029));
#75113=CARTESIAN_POINT('Ctrl Pts',(-20.8345254155557,-18.6883724788151,
-6.10697230589792));
#75114=CARTESIAN_POINT('Ctrl Pts',(-20.835474833797,-18.6960601175115,-6.10650442296411));
#75115=CARTESIAN_POINT('Ctrl Pts',(-20.835902697796,-18.6995980409213,-6.10628865262771));
#75116=CARTESIAN_POINT('Ctrl Pts',(-20.836848273354,-18.7075859868555,-6.10580048235774));
#75117=CARTESIAN_POINT('Ctrl Pts',(-20.837360790625,-18.7120365565819,-6.10552779540454));
#75118=CARTESIAN_POINT('Ctrl Pts',(-20.8388276184309,-18.7251399565725,
-6.10472296328847));
#75119=CARTESIAN_POINT('Ctrl Pts',(-20.8397426744963,-18.7337969628086,
-6.10418869001278));
#75120=CARTESIAN_POINT('Ctrl Pts',(-20.8458591842653,-18.7952888792466,
-6.10037679337727));
#75121=CARTESIAN_POINT('Ctrl Pts',(-20.8491244443308,-18.8482929538423,
-6.09700301862787));
#75122=CARTESIAN_POINT('Ctrl Pts',(-20.8507874982812,-18.9177948251246,
-6.09251065584329));
#75123=CARTESIAN_POINT('Ctrl Pts',(-20.8509892979677,-18.9342348571539,
-6.09144298497249));
#75124=CARTESIAN_POINT('Ctrl Pts',(-20.8510113339811,-18.9694500117011,
-6.08914723831414));
#75125=CARTESIAN_POINT('Ctrl Pts',(-20.8507733241541,-18.9882237924484,
-6.08791800906747));
#75126=CARTESIAN_POINT('Ctrl Pts',(-20.8462294472628,-19.1630893871222,
-6.07643127822385));
#75127=CARTESIAN_POINT('Ctrl Pts',(-20.8249136862804,-19.3182816586248,
-6.0660096583617));
#75128=CARTESIAN_POINT('Ctrl Pts',(-20.7855427580425,-19.4743833987669,
-6.05574893351126));
#75129=CARTESIAN_POINT('Ctrl Pts',(-20.7843514048602,-19.4790400558735,
-6.05544300635235));
#75130=CARTESIAN_POINT('Ctrl Pts',(-20.7672397017651,-19.5449885839064,
-6.05111271590937));
#75131=CARTESIAN_POINT('Ctrl Pts',(-20.7485917903037,-19.6055444826611,
-6.0471663605319));
#75132=CARTESIAN_POINT('Ctrl Pts',(-20.7257108607384,-19.6694941509089,
-6.04302907618597));
#75133=CARTESIAN_POINT('Ctrl Pts',(-20.7241527163644,-19.6738048039783,
-6.04275033647391));
#75134=CARTESIAN_POINT('Ctrl Pts',(-20.7225805821268,-19.6781103692884,
-6.04247206352563));
#75135=CARTESIAN_POINT('Origin',(-18.734,-18.952,0.));
#75136=CARTESIAN_POINT('',(-20.7225806512393,-19.6781101800117,-5.24452704027197));
#75137=CARTESIAN_POINT('',(-20.7225805821191,-19.6781103693095,-5.46434836675477));
#75138=CARTESIAN_POINT('',(-20.7225805821191,-19.6781103693095,0.));
#75139=CARTESIAN_POINT('',(-20.850999355781,-18.9536515516794,-5.51218507055412));
#75140=CARTESIAN_POINT('Ctrl Pts',(-20.7225805821191,-19.6781103693095,
-5.46434836675477));
#75141=CARTESIAN_POINT('Ctrl Pts',(-20.723192165304,-19.6764354415064,-5.46445566646443));
#75142=CARTESIAN_POINT('Ctrl Pts',(-20.7238016299532,-19.6747597476393,
-5.46456309084474));
#75143=CARTESIAN_POINT('Ctrl Pts',(-20.7256303769629,-19.6697118502574,
-5.46488693162053));
#75144=CARTESIAN_POINT('Ctrl Pts',(-20.7268431849093,-19.6663373843159,
-5.46510373048139));
#75145=CARTESIAN_POINT('Ctrl Pts',(-20.7294018383849,-19.6591610624263,
-5.46556547520601));
#75146=CARTESIAN_POINT('Ctrl Pts',(-20.7307453742014,-19.6553584966566,
-5.46581054749099));
#75147=CARTESIAN_POINT('Ctrl Pts',(-20.7343556019155,-19.645046875665,-5.4664761725672));
#75148=CARTESIAN_POINT('Ctrl Pts',(-20.7366013615508,-19.638530618166,-5.46689793361378));
#75149=CARTESIAN_POINT('Ctrl Pts',(-20.7477596008164,-19.6056334283903,
-5.46903245536519));
#75150=CARTESIAN_POINT('Ctrl Pts',(-20.7561823297465,-19.5790907753001,
-5.47077168259425));
#75151=CARTESIAN_POINT('Ctrl Pts',(-20.7792348623651,-19.5011441823547,
-5.47591306665285));
#75152=CARTESIAN_POINT('Ctrl Pts',(-20.7924441376168,-19.4493448821175,
-5.47937189794215));
#75153=CARTESIAN_POINT('Ctrl Pts',(-20.8350198964028,-19.2513733902427,
-5.4926211182554));
#75154=CARTESIAN_POINT('Ctrl Pts',(-20.8508830562357,-19.1027271546237,
-5.50259347648227));
#75155=CARTESIAN_POINT('Ctrl Pts',(-20.850999355781,-18.9536515516794,-5.51218507055412));
#75156=CARTESIAN_POINT('Ctrl Pts',(-20.8509993578165,-18.9536489404629,
-5.51218523856097));
#75157=CARTESIAN_POINT('Ctrl Pts',(-20.8510649773718,-18.8694029900064,
-5.51760566003188));
#75158=CARTESIAN_POINT('Ctrl Pts',(-20.8461018014202,-18.7852181728266,
-5.52290055521964));
#75159=CARTESIAN_POINT('Ctrl Pts',(-20.8349011934136,-18.6912099913197,
-5.52867294427367));
#75160=CARTESIAN_POINT('Ctrl Pts',(-20.8335940937956,-18.6808876607733,
-5.52930492195785));
#75161=CARTESIAN_POINT('Ctrl Pts',(-20.8312616502042,-18.6634977245725,
-5.53036658643347));
#75162=CARTESIAN_POINT('Ctrl Pts',(-20.8302765582527,-18.6564249915505,
-5.53079753558967));
#75163=CARTESIAN_POINT('Ctrl Pts',(-20.8283990621847,-18.6434267119139,
-5.5315880186461));
#75164=CARTESIAN_POINT('Ctrl Pts',(-20.827517252791,-18.6374997309757,-5.53194788389538));
#75165=CARTESIAN_POINT('Ctrl Pts',(-20.825646330153,-18.6252811756259,-5.53268858144462));
#75166=CARTESIAN_POINT('Ctrl Pts',(-20.824653965858,-18.6189901547168,-5.53306930663188));
#75167=CARTESIAN_POINT('Ctrl Pts',(-20.8223696973148,-18.6049219707014,
-5.53391930288454));
#75168=CARTESIAN_POINT('Ctrl Pts',(-20.8210627048583,-18.5971473268443,
-5.53438808989743));
#75169=CARTESIAN_POINT('Ctrl Pts',(-20.8176411993383,-18.5774675579438,
-5.5355723965986));
#75170=CARTESIAN_POINT('Ctrl Pts',(-20.815468048469,-18.5655728140616,-5.53628604971493));
#75171=CARTESIAN_POINT('Ctrl Pts',(-20.8024833837919,-18.497791162282,-5.5403413460611));
#75172=CARTESIAN_POINT('Ctrl Pts',(-20.7895226632367,-18.4423367872297,
-5.54361378928937));
#75173=CARTESIAN_POINT('Ctrl Pts',(-20.7635221180252,-18.3483650949568,
-5.54912160343954));
#75174=CARTESIAN_POINT('Ctrl Pts',(-20.7515805956661,-18.3095796629295,
-5.55138385254816));
#75175=CARTESIAN_POINT('Ctrl Pts',(-20.7072759613866,-18.1791378045608,
-5.55899523440277));
#75176=CARTESIAN_POINT('Ctrl Pts',(-20.6697202997907,-18.0893752959372,
-5.56423294202583));
#75177=CARTESIAN_POINT('Ctrl Pts',(-20.5749345088226,-17.900487267687,-5.575741133546));
#75178=CARTESIAN_POINT('Ctrl Pts',(-20.515576913746,-17.8027848451378,-5.5820144547951));
#75179=CARTESIAN_POINT('Ctrl Pts',(-20.441714467317,-17.7007846057636,-5.58944723154195));
#75180=CARTESIAN_POINT('Ctrl Pts',(-20.4347032415601,-17.6912711891749,
-5.59014960929642));
#75181=CARTESIAN_POINT('Ctrl Pts',(-20.4246086589607,-17.6778114606168,
-5.59115720652724));
#75182=CARTESIAN_POINT('Ctrl Pts',(-20.4215902367403,-17.6738164203315,
-5.59145803488116));
#75183=CARTESIAN_POINT('Ctrl Pts',(-20.4163586720484,-17.6669430045232,
-5.59197872083395));
#75184=CARTESIAN_POINT('Ctrl Pts',(-20.4141522225773,-17.6640595154036,
-5.59219810811991));
#75185=CARTESIAN_POINT('Ctrl Pts',(-20.4098553839566,-17.6584740426378,
-5.5926249521417));
#75186=CARTESIAN_POINT('Ctrl Pts',(-20.4077658687508,-17.6557714373895,
-5.59283234212935));
#75187=CARTESIAN_POINT('Ctrl Pts',(-20.4021012310066,-17.6484812580356,
-5.59339405878653));
#75188=CARTESIAN_POINT('Ctrl Pts',(-20.3985137604331,-17.6439033800854,
-5.59374925001738));
#75189=CARTESIAN_POINT('Ctrl Pts',(-20.3850731745406,-17.6268970135584,
-5.59507776404666));
#75190=CARTESIAN_POINT('Ctrl Pts',(-20.3750996332916,-17.6145649504899,
-5.59605916982759));
#75191=CARTESIAN_POINT('Ctrl Pts',(-20.2853517053845,-17.5061090604366,
-5.60484300666774));
#75192=CARTESIAN_POINT('Ctrl Pts',(-20.1973605142541,-17.4171179450614,
-5.61311310745137));
#75193=CARTESIAN_POINT('Ctrl Pts',(-20.0321701174072,-17.2772379764777,
-5.62741665042648));
#75194=CARTESIAN_POINT('Ctrl Pts',(-19.9585208567808,-17.222657833255,-5.63344658060375));
#75195=CARTESIAN_POINT('Ctrl Pts',(-19.8341707683413,-17.1424436807893,
-5.64296804818991));
#75196=CARTESIAN_POINT('Ctrl Pts',(-19.7855715780523,-17.1137758883874,
-5.64654257052223));
#75197=CARTESIAN_POINT('Ctrl Pts',(-19.7154818800429,-17.0761219158005,
-5.65149050811432));
#75198=CARTESIAN_POINT('Ctrl Pts',(-19.6949028474367,-17.0654976671957,
-5.65291918538296));
#75199=CARTESIAN_POINT('Ctrl Pts',(-19.6584462476372,-17.0474277527893,
-5.65540870699129));
#75200=CARTESIAN_POINT('Ctrl Pts',(-19.6426430670796,-17.039837842838,-5.65647446684823));
#75201=CARTESIAN_POINT('Ctrl Pts',(-19.6192400192665,-17.0289535487961,
-5.65803352456691));
#75202=CARTESIAN_POINT('Ctrl Pts',(-19.6117124894652,-17.0255062071014,
-5.65853209629923));
#75203=CARTESIAN_POINT('Ctrl Pts',(-19.5986006284094,-17.0195942434106,
-5.65939557996678));
#75204=CARTESIAN_POINT('Ctrl Pts',(-19.5930255428042,-17.0171094674979,
-5.65976118196537));
#75205=CARTESIAN_POINT('Ctrl Pts',(-19.5819064119512,-17.0122112805998,
-5.66048730988549));
#75206=CARTESIAN_POINT('Ctrl Pts',(-19.5763626196646,-17.0097974416917,
-5.66084784779554));
#75207=CARTESIAN_POINT('Ctrl Pts',(-19.5631489934511,-17.0041112764891,
-5.66170367722274));
#75208=CARTESIAN_POINT('Ctrl Pts',(-19.5554699804815,-17.0008604338197,
-5.6621982340119));
#75209=CARTESIAN_POINT('Ctrl Pts',(-19.5280515796337,-16.989443655501,-5.66395429549978));
#75210=CARTESIAN_POINT('Ctrl Pts',(-19.5082076248653,-16.9815310408094,
-5.6652072381635));
#75211=CARTESIAN_POINT('Ctrl Pts',(-19.3084660712501,-16.9053690997746,
-5.67764965640986));
#75212=CARTESIAN_POINT('Ctrl Pts',(-19.1201875471757,-16.8616474525009,
-5.68790565115474));
#75213=CARTESIAN_POINT('Ctrl Pts',(-18.8531492053921,-16.8369985791891,
-5.70254804019266));
#75214=CARTESIAN_POINT('Ctrl Pts',(-18.7774029112869,-16.8340901911473,
-5.70672656395101));
#75215=CARTESIAN_POINT('Ctrl Pts',(-18.6668516139817,-16.8357786704258,
-5.71305904194058));
#75216=CARTESIAN_POINT('Ctrl Pts',(-18.6320536306303,-16.8371694530356,
-5.71508642344316));
#75217=CARTESIAN_POINT('Ctrl Pts',(-18.5899319468194,-16.839894881452,-5.7175987823462));
#75218=CARTESIAN_POINT('Ctrl Pts',(-18.5825584452229,-16.8404107673196,
-5.71804074767399));
#75219=CARTESIAN_POINT('Ctrl Pts',(-18.5710565700527,-16.8412760475873,
-5.71873376464452));
#75220=CARTESIAN_POINT('Ctrl Pts',(-18.5669261816538,-16.8415989710012,
-5.71898335569992));
#75221=CARTESIAN_POINT('Ctrl Pts',(-18.5592408321956,-16.8422225327113,
-5.71944915900284));
#75222=CARTESIAN_POINT('Ctrl Pts',(-18.5556856738514,-16.8425200335916,
-5.71966519360376));
#75223=CARTESIAN_POINT('Ctrl Pts',(-18.5476150003735,-16.8432159474172,
-5.72015688339496));
#75224=CARTESIAN_POINT('Ctrl Pts',(-18.5431000230561,-16.8436198762006,
-5.72043284384559));
#75225=CARTESIAN_POINT('Ctrl Pts',(-18.5314073438093,-16.8447038182057,
-5.72114976964708));
#75226=CARTESIAN_POINT('Ctrl Pts',(-18.5242318248041,-16.84540599749,-5.72159193389962));
#75227=CARTESIAN_POINT('Ctrl Pts',(-18.4793497899922,-16.8500296306153,
-5.72437082687246));
#75228=CARTESIAN_POINT('Ctrl Pts',(-18.4417531864418,-16.8549264310823,
-5.72675693701609));
#75229=CARTESIAN_POINT('Ctrl Pts',(-18.2366588711491,-16.887261103057,-5.74002148790082));
#75230=CARTESIAN_POINT('Ctrl Pts',(-18.0727946768144,-16.9337567774534,
-5.75147113698783));
#75231=CARTESIAN_POINT('Ctrl Pts',(-17.8287253679685,-17.0359707178545,
-5.76866278538847));
#75232=CARTESIAN_POINT('Ctrl Pts',(-17.7437679165177,-17.0784645778304,
-5.77468924611025));
#75233=CARTESIAN_POINT('Ctrl Pts',(-17.6435447412113,-17.1373233536333,
-5.78182820053321));
#75234=CARTESIAN_POINT('Ctrl Pts',(-17.6253151209964,-17.1484030678603,
-5.78312834037129));
#75235=CARTESIAN_POINT('Ctrl Pts',(-17.5996365788949,-17.1645466103439,
-5.78496267368201));
#75236=CARTESIAN_POINT('Ctrl Pts',(-17.592048155024,-17.1693850727093,-5.78550512249112));
#75237=CARTESIAN_POINT('Ctrl Pts',(-17.5790118633132,-17.1778145607328,
-5.78643772774021));
#75238=CARTESIAN_POINT('Ctrl Pts',(-17.5735493637989,-17.1813826242763,
-5.78682873152825));
#75239=CARTESIAN_POINT('Ctrl Pts',(-17.5631229840833,-17.1882620328694,
-5.78757550937497));
#75240=CARTESIAN_POINT('Ctrl Pts',(-17.5581564458295,-17.1915692173964,
-5.78793143428601));
#75241=CARTESIAN_POINT('Ctrl Pts',(-17.5452805070876,-17.2002220176809,
-5.78885475186381));
#75242=CARTESIAN_POINT('Ctrl Pts',(-17.5373931075313,-17.2056002514883,
-5.78942090854513));
#75243=CARTESIAN_POINT('Ctrl Pts',(-17.510634010907,-17.224113053529,-5.79134384442678));
#75244=CARTESIAN_POINT('Ctrl Pts',(-17.4919396130848,-17.2375019103998,
-5.79269093324734));
#75245=CARTESIAN_POINT('Ctrl Pts',(-17.3325077768454,-17.3556629832336,
-5.80422227560228));
#75246=CARTESIAN_POINT('Ctrl Pts',(-17.2050834126516,-17.4772481249502,
-5.81365594412651));
#75247=CARTESIAN_POINT('Ctrl Pts',(-17.039077082204,-17.6805840586418,-5.82793846872569));
#75248=CARTESIAN_POINT('Ctrl Pts',(-16.9882547430038,-17.7513196534878,
-5.83270258609255));
#75249=CARTESIAN_POINT('Ctrl Pts',(-16.9217945585225,-17.8569970707073,
-5.83983014512697));
#75250=CARTESIAN_POINT('Ctrl Pts',(-16.90251926848,-17.889550985693,-5.84202747481105));
#75251=CARTESIAN_POINT('Ctrl Pts',(-16.8804458017486,-17.9292179267824,
-5.84472835267362));
#75252=CARTESIAN_POINT('Ctrl Pts',(-16.8767994796401,-17.9358540663859,
-5.84518097171932));
#75253=CARTESIAN_POINT('Ctrl Pts',(-16.8711945565141,-17.9461857171335,
-5.84588706220637));
#75254=CARTESIAN_POINT('Ctrl Pts',(-16.8692111317297,-17.9498677891718,
-5.84613898206746));
#75255=CARTESIAN_POINT('Ctrl Pts',(-16.8655578583016,-17.9566982047321,
-5.8466068642418));
#75256=CARTESIAN_POINT('Ctrl Pts',(-16.863885043555,-17.959844896381,-5.84682263465507));
#75257=CARTESIAN_POINT('Ctrl Pts',(-16.8601272308887,-17.9669568964184,
-5.84731080610661));
#75258=CARTESIAN_POINT('Ctrl Pts',(-16.8580468821083,-17.9709245852896,
-5.84758349417042));
#75259=CARTESIAN_POINT('Ctrl Pts',(-16.8519611864967,-17.9826214936684,
-5.84838833254776));
#75260=CARTESIAN_POINT('Ctrl Pts',(-16.8479909597664,-17.9903687410194,
-5.84892261102267));
#75261=CARTESIAN_POINT('Ctrl Pts',(-16.8201469732622,-18.0455374523063,
-5.85273461148439));
#75262=CARTESIAN_POINT('Ctrl Pts',(-16.7980188014963,-18.0938138114598,
-5.85610849055743));
#75263=CARTESIAN_POINT('Ctrl Pts',(-16.7705824356547,-18.1601476048199,
-5.86074703213836));
#75264=CARTESIAN_POINT('Ctrl Pts',(-16.7636640157269,-18.1775228680619,
-5.8619623206863));
#75265=CARTESIAN_POINT('Ctrl Pts',(-16.739913223645,-18.239550698721,-5.86629680707674));
#75266=CARTESIAN_POINT('Ctrl Pts',(-16.724361626426,-18.2846773929496,-5.8694426967701));
#75267=CARTESIAN_POINT('Ctrl Pts',(-16.6782280979619,-18.4348408869696,
-5.87981966685946));
#75268=CARTESIAN_POINT('Ctrl Pts',(-16.6542559121023,-18.5417322139677,
-5.88705182587264));
#75269=CARTESIAN_POINT('Ctrl Pts',(-16.6307922327491,-18.704530637206,-5.8976241297015));
#75270=CARTESIAN_POINT('Ctrl Pts',(-16.6250643057784,-18.7593473176632,
-5.90111265616119));
#75271=CARTESIAN_POINT('Ctrl Pts',(-16.6192506984924,-18.8485552851426,
-5.90666936732001));
#75272=CARTESIAN_POINT('Ctrl Pts',(-16.6178522138597,-18.8828322277822,
-5.90877597596377));
#75273=CARTESIAN_POINT('Ctrl Pts',(-16.6171091801909,-18.9279361511284,
-5.91151222463));
#75274=CARTESIAN_POINT('Ctrl Pts',(-16.6170139119708,-18.9387439941796,
-5.91216520000266));
#75275=CARTESIAN_POINT('Ctrl Pts',(-16.6169934394926,-18.9564501519871,
-5.91323066435871));
#75276=CARTESIAN_POINT('Ctrl Pts',(-16.6170191774154,-18.9633481119614,
-5.9136446825898));
#75277=CARTESIAN_POINT('Ctrl Pts',(-16.6171342791504,-18.9767024269151,
-5.91444419375255));
#75278=CARTESIAN_POINT('Ctrl Pts',(-16.6172194670201,-18.9831587327522,
-5.91482981298356));
#75279=CARTESIAN_POINT('Ctrl Pts',(-16.617484417735,-18.9980681579844,-5.91571825066866));
#75280=CARTESIAN_POINT('Ctrl Pts',(-16.6176852862598,-19.0065208283215,
-5.91622040297404));
#75281=CARTESIAN_POINT('Ctrl Pts',(-16.6183618793784,-19.0292564901604,
-5.91756707898111));
#75282=CARTESIAN_POINT('Ctrl Pts',(-16.6189316026856,-19.0435363987407,
-5.91840866081854));
#75283=CARTESIAN_POINT('Ctrl Pts',(-16.6254887723869,-19.1745657602676,
-5.92609439349616));
#75284=CARTESIAN_POINT('Ctrl Pts',(-16.6409925033073,-19.2906443606613,
-5.93262147566152));
#75285=CARTESIAN_POINT('Ctrl Pts',(-16.7008707918916,-19.5640784168669,
-5.94794486672316));
#75286=CARTESIAN_POINT('Ctrl Pts',(-16.7540025484123,-19.7187153940254,
-5.95655738493446));
#75287=CARTESIAN_POINT('Ctrl Pts',(-16.838239885856,-19.8947728879494,-5.96776743646225));
#75288=CARTESIAN_POINT('Ctrl Pts',(-16.8528070799986,-19.9235143187644,
-5.96964708166029));
#75289=CARTESIAN_POINT('Ctrl Pts',(-16.8714335886739,-19.958274062563,-5.97199523340606));
#75290=CARTESIAN_POINT('Ctrl Pts',(-16.8748761534455,-19.9646201880982,
-5.97242704984411));
#75291=CARTESIAN_POINT('Ctrl Pts',(-16.8803270273673,-19.9745469986074,
-5.97310760140977));
#75292=CARTESIAN_POINT('Ctrl Pts',(-16.8823134428908,-19.97813973093,-5.97335496039194));
#75293=CARTESIAN_POINT('Ctrl Pts',(-16.8860480084109,-19.9848481011705,
-5.97381884467594));
#75294=CARTESIAN_POINT('Ctrl Pts',(-16.8877935990292,-19.987965099636,-5.97403520622955));
#75295=CARTESIAN_POINT('Ctrl Pts',(-16.8917990286321,-19.9950750844817,
-5.97453060323972));
#75296=CARTESIAN_POINT('Ctrl Pts',(-16.8940639562644,-19.9990651387677,
-5.97480996282954));
#75297=CARTESIAN_POINT('Ctrl Pts',(-16.9000116291057,-20.0094640855736,
-5.97554149543378));
#75298=CARTESIAN_POINT('Ctrl Pts',(-16.9037149645511,-20.01586104459,-5.97599494777293));
#75299=CARTESIAN_POINT('Ctrl Pts',(-16.9282493267195,-20.0577332103697,
-5.97898511057316));
#75300=CARTESIAN_POINT('Ctrl Pts',(-16.9500756956761,-20.092611673444,-5.98157997802144));
#75301=CARTESIAN_POINT('Ctrl Pts',(-16.9785954782324,-20.135363514194,-5.98487201392494));
#75302=CARTESIAN_POINT('Ctrl Pts',(-16.9843504442667,-20.1438559761172,
-5.98553162334431));
#75303=CARTESIAN_POINT('Ctrl Pts',(-16.9905429064728,-20.1528525317468,
-5.98623618234779));
#75304=CARTESIAN_POINT('Ctrl Pts',(-16.9909192462669,-20.1533987372795,
-5.98627898093399));
#75305=CARTESIAN_POINT('Ctrl Pts',(-17.0042628851189,-20.1727457285681,
-5.98779574614873));
#75306=CARTESIAN_POINT('Ctrl Pts',(-17.0175330097642,-20.1913351602275,
-5.9892801694208));
#75307=CARTESIAN_POINT('Ctrl Pts',(-17.0582335406493,-20.2464425609985,
-5.99375508029232));
#75308=CARTESIAN_POINT('Ctrl Pts',(-17.0865472209864,-20.2822909156953,
-5.9967662323036));
#75309=CARTESIAN_POINT('Ctrl Pts',(-17.1865154855057,-20.4007713969403,
-6.00700650583097));
#75310=CARTESIAN_POINT('Ctrl Pts',(-17.2634088145626,-20.4787651800786,
-6.0142370854979));
#75311=CARTESIAN_POINT('Ctrl Pts',(-17.3875660103565,-20.5865753622057,
-6.02480607213136));
#75312=CARTESIAN_POINT('Ctrl Pts',(-17.4305385826985,-20.6210447137009,
-6.02829287176991));
#75313=CARTESIAN_POINT('Ctrl Pts',(-17.5023719924443,-20.6741954165705,
-6.03384715446885));
#75314=CARTESIAN_POINT('Ctrl Pts',(-17.5304270171886,-20.6939175907363,
-6.03595301961624));
#75315=CARTESIAN_POINT('Ctrl Pts',(-17.5679391609692,-20.7189487547639,
-6.03868845848497));
#75316=CARTESIAN_POINT('Ctrl Pts',(-17.5769741552405,-20.7248781637844,
-6.03934135028552));
#75317=CARTESIAN_POINT('Ctrl Pts',(-17.591849770131,-20.7344784513021,-6.04040671323086));
#75318=CARTESIAN_POINT('Ctrl Pts',(-17.5976635482948,-20.7381903726155,
-6.04082071306157));
#75319=CARTESIAN_POINT('Ctrl Pts',(-17.6089545765941,-20.745321913891,-6.04162021283985));
#75320=CARTESIAN_POINT('Ctrl Pts',(-17.6144295272225,-20.7487450151534,
-6.04200583896018));
#75321=CARTESIAN_POINT('Ctrl Pts',(-17.6271101523052,-20.7565928523384,
-6.04289432703066));
#75322=CARTESIAN_POINT('Ctrl Pts',(-17.6343268773118,-20.7609995920514,
-6.04339652258957));
#75323=CARTESIAN_POINT('Ctrl Pts',(-17.6538130468195,-20.7727387077009,
-6.0447433911984));
#75324=CARTESIAN_POINT('Ctrl Pts',(-17.6661308005046,-20.779990340027,-6.04558512105175));
#75325=CARTESIAN_POINT('Ctrl Pts',(-17.7800283110356,-20.8454991939601,
-6.05328251020523));
#75326=CARTESIAN_POINT('Ctrl Pts',(-17.8862102831229,-20.8953628239355,
-6.05981994772241));
#75327=CARTESIAN_POINT('Ctrl Pts',(-18.1493513218196,-20.9932374662671,
-6.07518832521485));
#75328=CARTESIAN_POINT('Ctrl Pts',(-18.3087952660216,-21.0323012183235,
-6.08383357512629));
#75329=CARTESIAN_POINT('Ctrl Pts',(-18.502352701236,-21.0565234722268,-6.09504693551604));
#75330=CARTESIAN_POINT('Ctrl Pts',(-18.5336629896907,-21.0597344140016,
-6.09688405070898));
#75331=CARTESIAN_POINT('Ctrl Pts',(-18.5721759019377,-21.0628181670366,
-6.0991848575549));
#75332=CARTESIAN_POINT('Ctrl Pts',(-18.5793232747794,-21.0633539448271,
-6.09961358317473));
#75333=CARTESIAN_POINT('Ctrl Pts',(-18.5905569848703,-21.0641386935524,
-6.10029033648786));
#75334=CARTESIAN_POINT('Ctrl Pts',(-18.5946416350763,-21.0644121295011,
-6.10053701332016));
#75335=CARTESIAN_POINT('Ctrl Pts',(-18.6022940450339,-21.0649021078387,
-6.10100032690858));
#75336=CARTESIAN_POINT('Ctrl Pts',(-18.6058615687777,-21.0651214630624,
-6.10121680421671));
#75337=CARTESIAN_POINT('Ctrl Pts',(-18.6140274954184,-21.0656028037622,
-6.10171340629773));
#75338=CARTESIAN_POINT('Ctrl Pts',(-18.6186261947882,-21.0658588169678,
-6.1019938612747));
#75339=CARTESIAN_POINT('Ctrl Pts',(-18.6328371901955,-21.0666034430593,
-6.10286289260626));
#75340=CARTESIAN_POINT('Ctrl Pts',(-18.6424518537548,-21.0670415041728,
-6.10345418875523));
#75341=CARTESIAN_POINT('Ctrl Pts',(-18.7385994139874,-21.0707653472408,
-6.10939834059158));
#75342=CARTESIAN_POINT('Ctrl Pts',(-18.8252445049579,-21.0688038923811,
-6.11500419074483));
#75343=CARTESIAN_POINT('Ctrl Pts',(-19.0379891875534,-21.0509017578764,
-6.12902183930854));
#75344=CARTESIAN_POINT('Ctrl Pts',(-19.1632601108586,-21.028905714308,-6.13748318541922));
#75345=CARTESIAN_POINT('Ctrl Pts',(-19.3790109779968,-20.9706554764984,
-6.15194737755517));
#75346=CARTESIAN_POINT('Ctrl Pts',(-19.4703936180671,-20.9391431933131,
-6.158042051408));
#75347=CARTESIAN_POINT('Ctrl Pts',(-19.5727827931087,-20.8957968620567,
-6.16482097640456));
#75348=CARTESIAN_POINT('Ctrl Pts',(-19.5861890752623,-20.889956813707,-6.1657077354927));
#75349=CARTESIAN_POINT('Ctrl Pts',(-19.6065883499041,-20.8808178562875,
-6.16705600375849));
#75350=CARTESIAN_POINT('Ctrl Pts',(-19.6136253670399,-20.8776188530583,
-6.16752091729008));
#75351=CARTESIAN_POINT('Ctrl Pts',(-19.6264196577487,-20.8717178433137,
-6.16836590062807));
#75352=CARTESIAN_POINT('Ctrl Pts',(-19.6321825539075,-20.8690283108749,
-6.16874639429736));
#75353=CARTESIAN_POINT('Ctrl Pts',(-19.644624186251,-20.8631534060413,-6.1695676512391));
#75354=CARTESIAN_POINT('Ctrl Pts',(-19.6512985340453,-20.8599588967214,
-6.17000809224879));
#75355=CARTESIAN_POINT('Ctrl Pts',(-19.6694152821869,-20.8511707302691,
-6.17120336567527));
#75356=CARTESIAN_POINT('Ctrl Pts',(-19.6808242886947,-20.8455086453087,
-6.17195581038795));
#75357=CARTESIAN_POINT('Ctrl Pts',(-19.7368646511553,-20.8170636582214,
-6.17565131416446));
#75358=CARTESIAN_POINT('Ctrl Pts',(-19.7807305318687,-20.7928030130521,
-6.17854200685107));
#75359=CARTESIAN_POINT('Ctrl Pts',(-19.9725202516072,-20.6776559891513,
-6.19124137582172));
#75360=CARTESIAN_POINT('Ctrl Pts',(-20.1097822700602,-20.5703460784515,
-6.2004348615193));
#75361=CARTESIAN_POINT('Ctrl Pts',(-20.2767028854959,-20.4030992219948,
-6.21342110654374));
#75362=CARTESIAN_POINT('Ctrl Pts',(-20.3190029979136,-20.3567723989518,
-6.21691359532654));
#75363=CARTESIAN_POINT('Ctrl Pts',(-20.3790003035009,-20.2848988890064,
-6.22229884916606));
#75364=CARTESIAN_POINT('Ctrl Pts',(-20.3982951711891,-20.2607271690287,
-6.2241048731261));
#75365=CARTESIAN_POINT('Ctrl Pts',(-20.421376504265,-20.2304757904981,-6.22637104482212));
#75366=CARTESIAN_POINT('Ctrl Pts',(-20.4256717695497,-20.2247868772316,
-6.22679745990223));
#75367=CARTESIAN_POINT('Ctrl Pts',(-20.4323832448442,-20.2158037990533,
-6.22747137329916));
#75368=CARTESIAN_POINT('Ctrl Pts',(-20.4348188361803,-20.2125240873201,
-6.22771753952508));
#75369=CARTESIAN_POINT('Ctrl Pts',(-20.4393684434147,-20.2063604976654,
-6.22818043108767));
#75370=CARTESIAN_POINT('Ctrl Pts',(-20.4414846510342,-20.2034783065243,
-6.22839700021274));
#75371=CARTESIAN_POINT('Ctrl Pts',(-20.4463180499241,-20.1968603275623,
-6.22889452790784));
#75372=CARTESIAN_POINT('Ctrl Pts',(-20.4490303145,-20.1931210088653,-6.22917582132584));
#75373=CARTESIAN_POINT('Ctrl Pts',(-20.457396701613,-20.1815067277241,-6.23004998870746));
#75374=CARTESIAN_POINT('Ctrl Pts',(-20.4630088913764,-20.173601911421,-6.23064562817186));
#75375=CARTESIAN_POINT('Ctrl Pts',(-20.5258583291827,-20.083777234927,-6.23741900611765));
#75376=CARTESIAN_POINT('Ctrl Pts',(-20.5772738357686,-19.9979506705685,
-6.24393193266537));
#75377=CARTESIAN_POINT('Ctrl Pts',(-20.6603886086506,-19.8339120813832,
-6.25604820103993));
#75378=CARTESIAN_POINT('Ctrl Pts',(-20.6938230701706,-19.7568678175932,
-6.26161635848641));
#75379=CARTESIAN_POINT('Ctrl Pts',(-20.722580459427,-19.6781107053232,-6.26710642520023));
#75380=CARTESIAN_POINT('',(-20.8509997150768,-18.9509016536907,-5.28730624892625));
#75381=CARTESIAN_POINT('Ctrl Pts',(-20.7225805821268,-19.6781103692884,
-6.04247206352563));
#75382=CARTESIAN_POINT('Ctrl Pts',(-20.7198613276793,-19.6855575244605,
-6.04199074651453));
#75383=CARTESIAN_POINT('Ctrl Pts',(-20.7171002195281,-19.6929894585156,
-6.04151082617329));
#75384=CARTESIAN_POINT('Ctrl Pts',(-20.711464594033,-19.7079014409026,-6.04054865701149));
#75385=CARTESIAN_POINT('Ctrl Pts',(-20.7085892401259,-19.715380995668,-6.04006644838188));
#75386=CARTESIAN_POINT('Ctrl Pts',(-20.7033484419158,-19.728785952518,-6.03920288357619));
#75387=CARTESIAN_POINT('Ctrl Pts',(-20.7009985599696,-19.7347172977286,
-6.03882101045798));
#75388=CARTESIAN_POINT('Ctrl Pts',(-20.6959422695857,-19.7473133163989,
-6.03801050624609));
#75389=CARTESIAN_POINT('Ctrl Pts',(-20.6932286285942,-19.753975014128,-6.03758212482112));
#75390=CARTESIAN_POINT('Ctrl Pts',(-20.6858431534448,-19.7718443371081,
-6.03643369174065));
#75391=CARTESIAN_POINT('Ctrl Pts',(-20.6811087182911,-19.7830259208666,
-6.03571576750528));
#75392=CARTESIAN_POINT('Ctrl Pts',(-20.657151087923,-19.8382791209533,-6.03217087236694));
#75393=CARTESIAN_POINT('Ctrl Pts',(-20.6365257003521,-19.8817296736474,
-6.02939218845373));
#75394=CARTESIAN_POINT('Ctrl Pts',(-20.5374257010067,-20.0733618598878,
-6.01711751652667));
#75395=CARTESIAN_POINT('Ctrl Pts',(-20.4430008541251,-20.2126007647328,
-6.00819945238123));
#75396=CARTESIAN_POINT('Ctrl Pts',(-20.268449046075,-20.4138139274042,-5.9936158203979));
#75397=CARTESIAN_POINT('Ctrl Pts',(-20.1986332455675,-20.4837565623116,
-5.98812314209123));
#75398=CARTESIAN_POINT('Ctrl Pts',(-20.1168931538418,-20.5549315393085,
-5.98170196872616));
#75399=CARTESIAN_POINT('Ctrl Pts',(-20.1095379797514,-20.5612477288602,
-5.98112423045765));
#75400=CARTESIAN_POINT('Ctrl Pts',(-20.0986146017065,-20.5704984797559,
-5.98026584768058));
#75401=CARTESIAN_POINT('Ctrl Pts',(-20.0950796393385,-20.5734723416122,
-5.97998800650598));
#75402=CARTESIAN_POINT('Ctrl Pts',(-20.0887912534957,-20.5787275264372,
-5.97949359408108));
#75403=CARTESIAN_POINT('Ctrl Pts',(-20.08604175398,-20.5810134686683,-5.97927736481212));
#75404=CARTESIAN_POINT('Ctrl Pts',(-20.0801385596345,-20.5858961615167,
-5.97881298399141));
#75405=CARTESIAN_POINT('Ctrl Pts',(-20.0769831836897,-20.5884907137006,
-5.97856468618755));
#75406=CARTESIAN_POINT('Ctrl Pts',(-20.068301446452,-20.5955873752138,-5.9778813537645));
#75407=CARTESIAN_POINT('Ctrl Pts',(-20.062759884528,-20.6000706829207,-5.97744500161648));
#75408=CARTESIAN_POINT('Ctrl Pts',(-20.033057799455,-20.6238534737716,-5.97510573783096));
#75409=CARTESIAN_POINT('Ctrl Pts',(-20.0085005799993,-20.6426487637712,
-5.97317005364767));
#75410=CARTESIAN_POINT('Ctrl Pts',(-19.9329337704002,-20.6979030235584,
-5.9672306842145));
#75411=CARTESIAN_POINT('Ctrl Pts',(-19.880709934652,-20.7326388686644,-5.96314956878737));
#75412=CARTESIAN_POINT('Ctrl Pts',(-19.7118261887119,-20.8344557117345,
-5.95019055033212));
#75413=CARTESIAN_POINT('Ctrl Pts',(-19.5902576457128,-20.8927760311196,
-5.94122489787439));
#75414=CARTESIAN_POINT('Ctrl Pts',(-19.4256424190388,-20.9532464318815,
-5.92993144791107));
#75415=CARTESIAN_POINT('Ctrl Pts',(-19.3869105031309,-20.9662156565853,
-5.92732950143879));
#75416=CARTESIAN_POINT('Ctrl Pts',(-19.3014162200389,-20.9921174902234,
-5.92171052523676));
#75417=CARTESIAN_POINT('Ctrl Pts',(-19.2545346195584,-21.0045800483641,
-5.9187089134785));
#75418=CARTESIAN_POINT('Ctrl Pts',(-19.1949880210372,-21.0182375587605,
-5.91499304460613));
#75419=CARTESIAN_POINT('Ctrl Pts',(-19.1826878316498,-21.0209434127713,
-5.91423057635414));
#75420=CARTESIAN_POINT('Ctrl Pts',(-19.1631556955338,-21.0250578029709,
-5.91302770587397));
#75421=CARTESIAN_POINT('Ctrl Pts',(-19.1559394285447,-21.0265385959881,
-5.912584998256));
#75422=CARTESIAN_POINT('Ctrl Pts',(-19.1424773013202,-21.0292279033673,
-5.91176223329126));
#75423=CARTESIAN_POINT('Ctrl Pts',(-19.1362334578543,-21.0304459855792,
-5.91138187425359));
#75424=CARTESIAN_POINT('Ctrl Pts',(-19.1223512322694,-21.0330893047646,
-5.9105389287685));
#75425=CARTESIAN_POINT('Ctrl Pts',(-19.1147102787907,-21.0345006746932,
-5.9100767889578));
#75426=CARTESIAN_POINT('Ctrl Pts',(-19.0924792252143,-21.0384805552392,
-5.90873741059866));
#75427=CARTESIAN_POINT('Ctrl Pts',(-19.0778695329014,-21.040938061153,-5.90786370346111));
#75428=CARTESIAN_POINT('Ctrl Pts',(-18.9612384320707,-21.0592998936367,
-5.90093809103395));
#75429=CARTESIAN_POINT('Ctrl Pts',(-18.8581971184174,-21.0678755262067,
-5.89512921233333));
#75430=CARTESIAN_POINT('Ctrl Pts',(-18.5952937615171,-21.0704748661084,
-5.88065398522196));
#75431=CARTESIAN_POINT('Ctrl Pts',(-18.436006941572,-21.0539912990993,-5.8722257145276));
#75432=CARTESIAN_POINT('Ctrl Pts',(-18.2326895487442,-21.0093606567924,
-5.86047064271721));
#75433=CARTESIAN_POINT('Ctrl Pts',(-18.1856551300218,-20.9973269068382,
-5.85767577255944));
#75434=CARTESIAN_POINT('Ctrl Pts',(-18.1316340607186,-20.9815084304755,
-5.85433394701235));
#75435=CARTESIAN_POINT('Ctrl Pts',(-18.1242003943299,-20.9792872591053,
-5.85387115419921));
#75436=CARTESIAN_POINT('Ctrl Pts',(-18.1123334864648,-20.9756702663182,
-5.85312741534205));
#75437=CARTESIAN_POINT('Ctrl Pts',(-18.1078922614552,-20.9743005957629,
-5.85284795639191));
#75438=CARTESIAN_POINT('Ctrl Pts',(-18.1000301583745,-20.9718475477278,
-5.85235121012464));
#75439=CARTESIAN_POINT('Ctrl Pts',(-18.0966074820963,-20.9707700845092,
-5.85213427132756));
#75440=CARTESIAN_POINT('Ctrl Pts',(-18.0893539546411,-20.9684663782786,
-5.85167304524102));
#75441=CARTESIAN_POINT('Ctrl Pts',(-18.0855239138788,-20.9672379372249,
-5.85142863566316));
#75442=CARTESIAN_POINT('Ctrl Pts',(-18.0751862144247,-20.9638897184746,
-5.85076663741833));
#75443=CARTESIAN_POINT('Ctrl Pts',(-18.0686853620824,-20.9617493060037,
-5.85034786238183));
#75444=CARTESIAN_POINT('Ctrl Pts',(-18.0363462607953,-20.9509275234716,
-5.84825266424105));
#75445=CARTESIAN_POINT('Ctrl Pts',(-18.0106682735654,-20.9417796446503,
-5.84655090551181));
#75446=CARTESIAN_POINT('Ctrl Pts',(-17.9367556887233,-20.9138282986456,
-5.84155567797127));
#75447=CARTESIAN_POINT('Ctrl Pts',(-17.8890268916447,-20.8937488226499,
-5.8382090057249));
#75448=CARTESIAN_POINT('Ctrl Pts',(-17.7166866316975,-20.8136876544287,
-5.82578742191394));
#75449=CARTESIAN_POINT('Ctrl Pts',(-17.5972859045534,-20.7432823710876,
-5.81654128797264));
#75450=CARTESIAN_POINT('Ctrl Pts',(-17.4531220622001,-20.6380184934663,
-5.80498306959785));
#75451=CARTESIAN_POINT('Ctrl Pts',(-17.4213206238985,-20.6133788836463,
-5.80240339928618));
#75452=CARTESIAN_POINT('Ctrl Pts',(-17.3446605537976,-20.5504067313845,
-5.79611643858223));
#75453=CARTESIAN_POINT('Ctrl Pts',(-17.3006635986976,-20.511075371361,-5.7924477674415));
#75454=CARTESIAN_POINT('Ctrl Pts',(-17.2495974566835,-20.4614328555569,
-5.78811126925235));
#75455=CARTESIAN_POINT('Ctrl Pts',(-17.2409054344102,-20.4528354620286,
-5.78737020289195));
#75456=CARTESIAN_POINT('Ctrl Pts',(-17.226702324861,-20.4385414638611,-5.78615421854932));
#75457=CARTESIAN_POINT('Ctrl Pts',(-17.2211479739558,-20.4328884344259,
-5.7856773888439));
#75458=CARTESIAN_POINT('Ctrl Pts',(-17.2111852191959,-20.4226341303159,
-5.78481969216978));
#75459=CARTESIAN_POINT('Ctrl Pts',(-17.2067656191817,-20.4180439111116,
-5.78443833715607));
#75460=CARTESIAN_POINT('Ctrl Pts',(-17.1973608827445,-20.4081874214596,
-5.78362492011295));
#75461=CARTESIAN_POINT('Ctrl Pts',(-17.1923819338307,-20.4029153397648,
-5.78319312868977));
#75462=CARTESIAN_POINT('Ctrl Pts',(-17.1789583927564,-20.3885543895332,
-5.78202574705693));
#75463=CARTESIAN_POINT('Ctrl Pts',(-17.1705663641182,-20.3794166141702,
-5.78129240919149));
#75464=CARTESIAN_POINT('Ctrl Pts',(-17.1277906707188,-20.3320098848024,
-5.77753527178085));
#75465=CARTESIAN_POINT('Ctrl Pts',(-17.0947282909668,-20.2925687542299,
-5.77456717922136));
#75466=CARTESIAN_POINT('Ctrl Pts',(-16.9574786046277,-20.1161587534877,
-5.76188221478874));
#75467=CARTESIAN_POINT('Ctrl Pts',(-16.8687774004017,-19.9679914318969,
-5.75276386095583));
#75468=CARTESIAN_POINT('Ctrl Pts',(-16.7622678956206,-19.7279862790549,
-5.73833990504607));
#75469=CARTESIAN_POINT('Ctrl Pts',(-16.7309001330982,-19.6429913259418,
-5.73327612219215));
#75470=CARTESIAN_POINT('Ctrl Pts',(-16.7023135357154,-19.5470062078873,
-5.72734232094472));
#75471=CARTESIAN_POINT('Ctrl Pts',(-16.6996202589123,-19.5377314552345,
-5.7267667652014));
#75472=CARTESIAN_POINT('Ctrl Pts',(-16.6957347023549,-19.5240007430237,
-5.72591101727965));
#75473=CARTESIAN_POINT('Ctrl Pts',(-16.6944933295053,-19.5195586433914,
-5.72563360367855));
#75474=CARTESIAN_POINT('Ctrl Pts',(-16.6923155684646,-19.5116663849891,
-5.72513966287343));
#75475=CARTESIAN_POINT('Ctrl Pts',(-16.6913733927432,-19.5082178741954,
-5.72492347522903));
#75476=CARTESIAN_POINT('Ctrl Pts',(-16.6893720889957,-19.5008191242431,
-5.72445885615565));
#75477=CARTESIAN_POINT('Ctrl Pts',(-16.6883156872461,-19.4968682570044,
-5.72421027676385));
#75478=CARTESIAN_POINT('Ctrl Pts',(-16.6854441713462,-19.4860029229224,
-5.72352539355565));
#75479=CARTESIAN_POINT('Ctrl Pts',(-16.6836526419961,-19.4790823588084,
-5.72308776244723));
#75480=CARTESIAN_POINT('Ctrl Pts',(-16.6742279538407,-19.4419001464867,
-5.72072948001408));
#75481=CARTESIAN_POINT('Ctrl Pts',(-16.6672300736544,-19.4114832617611,
-5.71877543470159));
#75482=CARTESIAN_POINT('Ctrl Pts',(-16.6277110565621,-19.2204787233204,
-5.7063968597271));
#75483=CARTESIAN_POINT('Ctrl Pts',(-16.6132534093868,-19.0567262630695,
-5.69536058959103));
#75484=CARTESIAN_POINT('Ctrl Pts',(-16.6210919675133,-18.7758322166447,
-5.67700329075265));
#75485=CARTESIAN_POINT('Ctrl Pts',(-16.6340766898099,-18.6591768353486,
-5.6695392360968));
#75486=CARTESIAN_POINT('Ctrl Pts',(-16.6594065810645,-18.530152324898,-5.66151057757297));
#75487=CARTESIAN_POINT('Ctrl Pts',(-16.6623022073903,-18.5161541709416,
-5.66064232264771));
#75488=CARTESIAN_POINT('Ctrl Pts',(-16.6671361131119,-18.4939233971635,
-5.65926765737429));
#75489=CARTESIAN_POINT('Ctrl Pts',(-16.6689822908034,-18.4856713981177,
-5.65875831659285));
#75490=CARTESIAN_POINT('Ctrl Pts',(-16.6723253377142,-18.4711379835352,
-5.6578628452105));
#75491=CARTESIAN_POINT('Ctrl Pts',(-16.6738015868424,-18.464851981585,-5.65747605805226));
#75492=CARTESIAN_POINT('Ctrl Pts',(-16.6769142498729,-18.4518652257022,
-5.65667800713446));
#75493=CARTESIAN_POINT('Ctrl Pts',(-16.678554700752,-18.4451655108729,-5.65626687853038));
#75494=CARTESIAN_POINT('Ctrl Pts',(-16.6828491740303,-18.4279903974839,
-5.65521434301624));
#75495=CARTESIAN_POINT('Ctrl Pts',(-16.685550733427,-18.4175270042033,-5.65457447640615));
#75496=CARTESIAN_POINT('Ctrl Pts',(-16.6971570196483,-18.3739558282852,
-5.65191519260697));
#75497=CARTESIAN_POINT('Ctrl Pts',(-16.7067855018262,-18.3410450379083,
-5.64991927298028));
#75498=CARTESIAN_POINT('Ctrl Pts',(-16.7339485491348,-18.2559291679024,
-5.64477901105708));
#75499=CARTESIAN_POINT('Ctrl Pts',(-16.7527281729848,-18.2041477412728,
-5.64167398117025));
#75500=CARTESIAN_POINT('Ctrl Pts',(-16.8147534794709,-18.0519278133802,
-5.63253398323416));
#75501=CARTESIAN_POINT('Ctrl Pts',(-16.8637797234717,-17.9540450145168,
-5.62664775917396));
#75502=CARTESIAN_POINT('Ctrl Pts',(-16.9416255080197,-17.8246943657777,
-5.61842857635207));
#75503=CARTESIAN_POINT('Ctrl Pts',(-16.964153940979,-17.7896450327833,-5.61615173333929));
#75504=CARTESIAN_POINT('Ctrl Pts',(-17.0311691688804,-17.6918535530327,
-5.60959402237034));
#75505=CARTESIAN_POINT('Ctrl Pts',(-17.0780562126549,-17.6308454345246,
-5.60525295951788));
#75506=CARTESIAN_POINT('Ctrl Pts',(-17.1343452729096,-17.5653190284406,
-5.60013340262089));
#75507=CARTESIAN_POINT('Ctrl Pts',(-17.1405878546146,-17.5581502627241,
-5.59956679206036));
#75508=CARTESIAN_POINT('Ctrl Pts',(-17.1499110353158,-17.5475883251614,
-5.59872185141719));
#75509=CARTESIAN_POINT('Ctrl Pts',(-17.1529548136374,-17.54416260945,-5.5984461995367));
#75510=CARTESIAN_POINT('Ctrl Pts',(-17.1583908761751,-17.5380842852842,
-5.59795419332101));
#75511=CARTESIAN_POINT('Ctrl Pts',(-17.1607787746501,-17.535427822072,-5.59773816856348));
#75512=CARTESIAN_POINT('Ctrl Pts',(-17.1659280394438,-17.5297285033819,
-5.59727252853963));
#75513=CARTESIAN_POINT('Ctrl Pts',(-17.1686915042528,-17.5266876847324,
-5.59702275810791));
#75514=CARTESIAN_POINT('Ctrl Pts',(-17.1763461053308,-17.5183139437054,
-5.59633130563363));
#75515=CARTESIAN_POINT('Ctrl Pts',(-17.1812557056297,-17.5129980832504,
-5.59588825459382));
#75516=CARTESIAN_POINT('Ctrl Pts',(-17.2083373842509,-17.4839754087953,
-5.59344728684747));
#75517=CARTESIAN_POINT('Ctrl Pts',(-17.2310239128924,-17.4607571520029,
-5.59141320372699));
#75518=CARTESIAN_POINT('Ctrl Pts',(-17.3706342740981,-17.3242971697599,
-5.57900885727586));
#75519=CARTESIAN_POINT('Ctrl Pts',(-17.4997640738172,-17.2243298334111,
-5.56804743882401));
#75520=CARTESIAN_POINT('Ctrl Pts',(-17.739058298427,-17.0797210381389,-5.54978433289827));
#75521=CARTESIAN_POINT('Ctrl Pts',(-17.8438879987841,-17.0276700036513,
-5.54234245908303));
#75522=CARTESIAN_POINT('Ctrl Pts',(-17.9657765590723,-16.9792541960539,
-5.53433428229327));
#75523=CARTESIAN_POINT('Ctrl Pts',(-17.9791124357856,-16.9741127324091,
-5.53346614086503));
#75524=CARTESIAN_POINT('Ctrl Pts',(-18.0004192888552,-16.9661450626522,
-5.53209162075742));
#75525=CARTESIAN_POINT('Ctrl Pts',(-18.0083567183911,-16.9632309528131,
-5.53158231260737));
#75526=CARTESIAN_POINT('Ctrl Pts',(-18.0223859693702,-16.9581754936131,
-5.53068687918324));
#75527=CARTESIAN_POINT('Ctrl Pts',(-18.0284704879456,-16.956014328731,-5.53030009752698));
#75528=CARTESIAN_POINT('Ctrl Pts',(-18.0410752470856,-16.9516020731792,
-5.52950203937665));
#75529=CARTESIAN_POINT('Ctrl Pts',(-18.0475968000327,-16.9493549421735,
-5.5290908981296));
#75530=CARTESIAN_POINT('Ctrl Pts',(-18.0643640190189,-16.9436689892503,
-5.52803829178658));
#75531=CARTESIAN_POINT('Ctrl Pts',(-18.0746253254795,-16.9402766490095,
-5.52739836739773));
#75532=CARTESIAN_POINT('Ctrl Pts',(-18.1175532159352,-16.9264486323259,
-5.52473852225137));
#75533=CARTESIAN_POINT('Ctrl Pts',(-18.1504460339223,-16.9167285326677,
-5.52274211172097));
#75534=CARTESIAN_POINT('Ctrl Pts',(-18.2367448549157,-16.8934908737408,
-5.51760029990378));
#75535=CARTESIAN_POINT('Ctrl Pts',(-18.2904687928593,-16.8812505668078,
-5.51449424212405));
#75536=CARTESIAN_POINT('Ctrl Pts',(-18.4520702392655,-16.8510106601424,
-5.50535245073789));
#75537=CARTESIAN_POINT('Ctrl Pts',(-18.5609275332916,-16.8392559540426,
-5.49946545520543));
#75538=CARTESIAN_POINT('Ctrl Pts',(-18.7135737336649,-16.8346539491919,
-5.49115109301115));
#75539=CARTESIAN_POINT('Ctrl Pts',(-18.7569710264611,-16.8346800745713,
-5.48877924591538));
#75540=CARTESIAN_POINT('Ctrl Pts',(-18.8292972566213,-16.8369475101901,
-5.48477243494056));
#75541=CARTESIAN_POINT('Ctrl Pts',(-18.8582363099455,-16.8384499454004,
-5.48315476497162));
#75542=CARTESIAN_POINT('Ctrl Pts',(-18.9346302399487,-16.8439904591386,
-5.4788257899165));
#75543=CARTESIAN_POINT('Ctrl Pts',(-18.9819924562815,-16.8490364456496,
-5.47608199229976));
#75544=CARTESIAN_POINT('Ctrl Pts',(-19.0367858363314,-16.8567507661122,
-5.47279662993194));
#75545=CARTESIAN_POINT('Ctrl Pts',(-19.0444254167679,-16.8578689937587,
-5.47233604094988));
#75546=CARTESIAN_POINT('Ctrl Pts',(-19.0566426431864,-16.8597255859386,
-5.47159517480974));
#75547=CARTESIAN_POINT('Ctrl Pts',(-19.0612243583322,-16.8604372547504,
-5.47131636665814));
#75548=CARTESIAN_POINT('Ctrl Pts',(-19.0693462033892,-16.8617261448277,
-5.47082035706679));
#75549=CARTESIAN_POINT('Ctrl Pts',(-19.0728872470253,-16.8622973179467,
-5.4706035005397));
#75550=CARTESIAN_POINT('Ctrl Pts',(-19.0804023027107,-16.8635291064289,
-5.4701419743159));
#75551=CARTESIAN_POINT('Ctrl Pts',(-19.08437582362,-16.8641920561954,-5.4698971799282));
#75552=CARTESIAN_POINT('Ctrl Pts',(-19.0951226615497,-16.8660166226016,
-5.4692330761317));
#75553=CARTESIAN_POINT('Ctrl Pts',(-19.1018921854005,-16.8671998742338,
-5.468812567668));
#75554=CARTESIAN_POINT('Ctrl Pts',(-19.1358176007472,-16.873300108826,-5.46669464178307));
#75555=CARTESIAN_POINT('Ctrl Pts',(-19.1628799077318,-16.8787145692043,
-5.46497123826257));
#75556=CARTESIAN_POINT('Ctrl Pts',(-19.2413208806372,-16.8960099601536,
-5.45989180490496));
#75557=CARTESIAN_POINT('Ctrl Pts',(-19.292369163295,-16.9092830237788,-5.4564805846112));
#75558=CARTESIAN_POINT('Ctrl Pts',(-19.4893962962023,-16.9684493731692,
-5.443025941233));
#75559=CARTESIAN_POINT('Ctrl Pts',(-19.630743738301,-17.028213400295,-5.43278495773439));
#75560=CARTESIAN_POINT('Ctrl Pts',(-19.8351666165557,-17.1421157417419,
-5.41775117662028));
#75561=CARTESIAN_POINT('Ctrl Pts',(-19.9036042009194,-17.1855692257347,
-5.41266576978646));
#75562=CARTESIAN_POINT('Ctrl Pts',(-19.9802494915794,-17.2406467292543,
-5.40690975551563));
#75563=CARTESIAN_POINT('Ctrl Pts',(-19.9910345962073,-17.248552950817,-5.40609821615784));
#75564=CARTESIAN_POINT('Ctrl Pts',(-20.0082998157767,-17.2614628123634,
-5.40479630893277));
#75565=CARTESIAN_POINT('Ctrl Pts',(-20.0148269539294,-17.2664026814517,
-5.40430347382937));
#75566=CARTESIAN_POINT('Ctrl Pts',(-20.0262667052871,-17.2751653314715,
-5.4034385049794));
#75567=CARTESIAN_POINT('Ctrl Pts',(-20.0311913849779,-17.2789721295821,
-5.40306574858598));
#75568=CARTESIAN_POINT('Ctrl Pts',(-20.0414189170293,-17.28695036271,-5.40229074539027));
#75569=CARTESIAN_POINT('Ctrl Pts',(-20.046718767995,-17.2911255444738,-5.40188865314042));
#75570=CARTESIAN_POINT('Ctrl Pts',(-20.0603035781497,-17.301933199629,-5.40085666677675));
#75571=CARTESIAN_POINT('Ctrl Pts',(-20.0685588512478,-17.3086028155483,
-5.40022826594452));
#75572=CARTESIAN_POINT('Ctrl Pts',(-20.0864173484392,-17.3232543981682,
-5.39886583046651));
#75573=CARTESIAN_POINT('Ctrl Pts',(-20.0960008459766,-17.331259852644,-5.39813276376099));
#75574=CARTESIAN_POINT('Ctrl Pts',(-20.1235847797125,-17.3547192027848,
-5.39601658069598));
#75575=CARTESIAN_POINT('Ctrl Pts',(-20.1413973090868,-17.3703917415524,
-5.39464226554776));
#75576=CARTESIAN_POINT('Ctrl Pts',(-20.2021281744288,-17.425665033814,-5.38992380358323));
#75577=CARTESIAN_POINT('Ctrl Pts',(-20.2436705206517,-17.4667409547304,
-5.38663873181035));
#75578=CARTESIAN_POINT('Ctrl Pts',(-20.3969219790516,-17.6313544932354,
-5.37416526857529));
#75579=CARTESIAN_POINT('Ctrl Pts',(-20.4955963124143,-17.7661729973952,
-5.36539600128428));
#75580=CARTESIAN_POINT('Ctrl Pts',(-20.6055540151064,-17.9609190737075,
-5.35285736722032));
#75581=CARTESIAN_POINT('Ctrl Pts',(-20.6316259216043,-18.0118029633074,
-5.34958651530647));
#75582=CARTESIAN_POINT('Ctrl Pts',(-20.6593252176873,-18.0717214043159,
-5.34567035599239));
#75583=CARTESIAN_POINT('Ctrl Pts',(-20.6629947229612,-18.0797919098864,
-5.34514155844039));
#75584=CARTESIAN_POINT('Ctrl Pts',(-20.6684560496856,-18.0920062954349,
-5.34433890238172));
#75585=CARTESIAN_POINT('Ctrl Pts',(-20.670285537329,-18.0961333648752,-5.34406729485529));
#75586=CARTESIAN_POINT('Ctrl Pts',(-20.673536575191,-18.1035310311175,-5.34357967327026));
#75587=CARTESIAN_POINT('Ctrl Pts',(-20.6749630741608,-18.1067993953323,
-5.34336396583261));
#75588=CARTESIAN_POINT('Ctrl Pts',(-20.6780343512004,-18.1138850212355,
-5.34289572459172));
#75589=CARTESIAN_POINT('Ctrl Pts',(-20.6796761250838,-18.1177034748547,
-5.34264301807798));
#75590=CARTESIAN_POINT('Ctrl Pts',(-20.6842304188109,-18.1283824531688,
-5.34193529686528));
#75591=CARTESIAN_POINT('Ctrl Pts',(-20.6871179358036,-18.1352534818269,
-5.34147880744297));
#75592=CARTESIAN_POINT('Ctrl Pts',(-20.7036702204672,-18.1752304365363,
-5.33881692638574));
#75593=CARTESIAN_POINT('Ctrl Pts',(-20.7165285144512,-18.2086615378309,
-5.33656739661333));
#75594=CARTESIAN_POINT('Ctrl Pts',(-20.7551281736653,-18.3171568528273,
-5.32922798578443));
#75595=CARTESIAN_POINT('Ctrl Pts',(-20.7774988580308,-18.3933447911045,
-5.32401735506563));
#75596=CARTESIAN_POINT('Ctrl Pts',(-20.8323034292351,-18.628040232454,-5.30810742997659));
#75597=CARTESIAN_POINT('Ctrl Pts',(-20.8509158166609,-18.7891922537898,
-5.2974224999678));
#75598=CARTESIAN_POINT('Ctrl Pts',(-20.8509997150768,-18.9509016536907,
-5.28730624892625));
#75599=CARTESIAN_POINT('Ctrl Pts',(-20.8509997162491,-18.9509039154662,
-5.28730610743365));
#75600=CARTESIAN_POINT('Ctrl Pts',(-20.8510131380821,-18.9768271137295,
-5.28568439929136));
#75601=CARTESIAN_POINT('Ctrl Pts',(-20.8505504063414,-19.0027494389046,
-5.28407670778165));
#75602=CARTESIAN_POINT('Ctrl Pts',(-20.8489736679247,-19.0462644244691,
-5.28140093350177));
#75603=CARTESIAN_POINT('Ctrl Pts',(-20.8481159279852,-19.0638627293641,
-5.28032511708845));
#75604=CARTESIAN_POINT('Ctrl Pts',(-20.8465415703195,-19.0895615458405,
-5.27876302123768));
#75605=CARTESIAN_POINT('Ctrl Pts',(-20.8459978383086,-19.0976715452308,
-5.2782713554403));
#75606=CARTESIAN_POINT('Ctrl Pts',(-20.8449526635068,-19.1120220081581,
-5.27740361134384));
#75607=CARTESIAN_POINT('Ctrl Pts',(-20.844470224362,-19.1182637184008,-5.27702694083171));
#75608=CARTESIAN_POINT('Ctrl Pts',(-20.843461131979,-19.1306063535202,-5.27628355624966));
#75609=CARTESIAN_POINT('Ctrl Pts',(-20.842935681016,-19.1367073128147,-5.27591680815732));
#75610=CARTESIAN_POINT('Ctrl Pts',(-20.8418361314369,-19.1488572085538,
-5.27518781569256));
#75611=CARTESIAN_POINT('Ctrl Pts',(-20.8412624478398,-19.1549061227731,
-5.27482556195104));
#75612=CARTESIAN_POINT('Ctrl Pts',(-20.8398285560976,-19.1693626419309,
-5.2739613853597));
#75613=CARTESIAN_POINT('Ctrl Pts',(-20.838944023514,-19.1777677718445,-5.27346023124555));
#75614=CARTESIAN_POINT('Ctrl Pts',(-20.8360988468823,-19.2033318591447,
-5.27193973537557));
#75615=CARTESIAN_POINT('Ctrl Pts',(-20.8339785147008,-19.2204725858573,
-5.27092540743934));
#75616=CARTESIAN_POINT('Ctrl Pts',(-20.8260337998877,-19.2788270918117,
-5.26748809935229));
#75617=CARTESIAN_POINT('Ctrl Pts',(-20.8192037229416,-19.319895539757,-5.26509636444063));
#75618=CARTESIAN_POINT('Ctrl Pts',(-20.7899098998943,-19.4687639214598,
-5.25649244291624));
#75619=CARTESIAN_POINT('Ctrl Pts',(-20.7602778622481,-19.5748697263155,
-5.25049681220908));
#75620=CARTESIAN_POINT('Ctrl Pts',(-20.7225806512393,-19.6781101800116,
-5.24452704027197));
#75621=CARTESIAN_POINT('Origin',(-18.734,-18.952,0.));
#75622=CARTESIAN_POINT('',(-20.7225805839746,-19.678110364228,-4.44630500845844));
#75623=CARTESIAN_POINT('',(-20.7225805678527,-19.6781104083805,-4.66702139913379));
#75624=CARTESIAN_POINT('',(-20.7225805821191,-19.6781103693095,0.));
#75625=CARTESIAN_POINT('Ctrl Pts',(-20.7225805678527,-19.6781104083805,
-4.66702139913379));
#75626=CARTESIAN_POINT('Ctrl Pts',(-20.7691765609132,-19.550499117769,-4.67446203916752));
#75627=CARTESIAN_POINT('Ctrl Pts',(-20.8033897580608,-19.4186748613786,
-4.68169555986857));
#75628=CARTESIAN_POINT('Ctrl Pts',(-20.830945610111,-19.2453826582096,-4.69152890075376));
#75629=CARTESIAN_POINT('Ctrl Pts',(-20.8360618100052,-19.2061457370852,
-4.69377787057993));
#75630=CARTESIAN_POINT('Ctrl Pts',(-20.8416060206598,-19.1517834556233,
-4.69695251884968));
#75631=CARTESIAN_POINT('Ctrl Pts',(-20.842976080738,-19.1367604708237,-4.69783600284219));
#75632=CARTESIAN_POINT('Ctrl Pts',(-20.8450676748484,-19.1107556837715,
-4.69937794229532));
#75633=CARTESIAN_POINT('Ctrl Pts',(-20.8458643547855,-19.0997803445484,
-4.7000326018113));
#75634=CARTESIAN_POINT('Ctrl Pts',(-20.8468897381308,-19.0839455008159,
-4.70098335630389));
#75635=CARTESIAN_POINT('Ctrl Pts',(-20.8471873278431,-19.0790904286316,
-4.70127570854314));
#75636=CARTESIAN_POINT('Ctrl Pts',(-20.8476764826095,-19.0706328030768,
-4.70178652843945));
#75637=CARTESIAN_POINT('Ctrl Pts',(-20.8478755777288,-19.0670306778501,
-4.70200457442121));
#75638=CARTESIAN_POINT('Ctrl Pts',(-20.8482735902435,-19.0594793970784,
-4.70246271750475));
#75639=CARTESIAN_POINT('Ctrl Pts',(-20.8484706504419,-19.0555302034396,
-4.70270291271344));
#75640=CARTESIAN_POINT('Ctrl Pts',(-20.8489642020017,-19.0450493172144,
-4.70334190839892));
#75641=CARTESIAN_POINT('Ctrl Pts',(-20.8492414963038,-19.038516824435,-4.70374176028672));
#75642=CARTESIAN_POINT('Ctrl Pts',(-20.8502933311571,-19.0106966931555,
-4.70545104988098));
#75643=CARTESIAN_POINT('Ctrl Pts',(-20.8507767750839,-18.9894001258531,
-4.70677554117578));
#75644=CARTESIAN_POINT('Ctrl Pts',(-20.8509781231563,-18.9629269108544,
-4.70843890180712));
#75645=CARTESIAN_POINT('Ctrl Pts',(-20.8509985064309,-18.9577528859984,
-4.70876479897971));
#75646=CARTESIAN_POINT('Ctrl Pts',(-20.8510131829577,-18.9040721336999,
-4.71215398694898));
#75647=CARTESIAN_POINT('Ctrl Pts',(-20.8493592892078,-18.8555823858534,
-4.71528283048994));
#75648=CARTESIAN_POINT('Ctrl Pts',(-20.8326138632352,-18.6113421565125,
-4.73125354343386));
#75649=CARTESIAN_POINT('Ctrl Pts',(-20.7920024717649,-18.4182599620961,
-4.74444618606871));
#75650=CARTESIAN_POINT('Ctrl Pts',(-20.7092042437438,-18.1887683984147,
-4.75978168055878));
#75651=CARTESIAN_POINT('Ctrl Pts',(-20.6915454806286,-18.144553069643,-4.76272646534576));
#75652=CARTESIAN_POINT('Ctrl Pts',(-20.6673796253022,-18.0895101133125,
-4.76638241527231));
#75653=CARTESIAN_POINT('Ctrl Pts',(-20.6622477601342,-18.078097164296,-4.7671399405995));
#75654=CARTESIAN_POINT('Ctrl Pts',(-20.6539422309451,-18.0600555950774,
-4.76833676900666));
#75655=CARTESIAN_POINT('Ctrl Pts',(-20.6508347867218,-18.0533969763163,
-4.76877833878035));
#75656=CARTESIAN_POINT('Ctrl Pts',(-20.6449719414798,-18.041002895943,-4.76960003552102));
#75657=CARTESIAN_POINT('Ctrl Pts',(-20.6422252369273,-18.0352634341076,
-4.76998045774046));
#75658=CARTESIAN_POINT('Ctrl Pts',(-20.6360566854916,-18.0225215950203,
-4.77082485155876));
#75659=CARTESIAN_POINT('Ctrl Pts',(-20.6326219512864,-18.0155255322615,
-4.77128836875544));
#75660=CARTESIAN_POINT('Ctrl Pts',(-20.6224963088177,-17.9951857501949,
-4.77263575676896));
#75661=CARTESIAN_POINT('Ctrl Pts',(-20.6157027231138,-17.9818934615505,
-4.77351603000565));
#75662=CARTESIAN_POINT('Ctrl Pts',(-20.5587597163249,-17.8733282758606,
-4.78070606476363));
#75663=CARTESIAN_POINT('Ctrl Pts',(-20.5015468641977,-17.7819302471413,
-4.78675002458835));
#75664=CARTESIAN_POINT('Ctrl Pts',(-20.3582472358736,-17.587673189725,-4.80001576019911));
#75665=CARTESIAN_POINT('Ctrl Pts',(-20.268862992358,-17.4878417496967,-4.80713451610839));
#75666=CARTESIAN_POINT('Ctrl Pts',(-20.1586113012438,-17.3859728591617,
-4.81548043959687));
#75667=CARTESIAN_POINT('Ctrl Pts',(-20.1464278923326,-17.3749756517987,
-4.81639768451699));
#75668=CARTESIAN_POINT('Ctrl Pts',(-20.0943136527319,-17.329023719481,-4.82030605725783));
#75669=CARTESIAN_POINT('Ctrl Pts',(-20.0532070431934,-17.2954381951771,
-4.82335179591882));
#75670=CARTESIAN_POINT('Ctrl Pts',(-20.0039435818771,-17.2581853521563,
-4.82701711043678));
#75671=CARTESIAN_POINT('Ctrl Pts',(-19.9969687793924,-17.2529783348072,
-4.82753639671103));
#75672=CARTESIAN_POINT('Ctrl Pts',(-19.9863559862622,-17.2451568461038,
-4.82832739005602));
#75673=CARTESIAN_POINT('Ctrl Pts',(-19.9827413826037,-17.2425105946938,
-4.82859694230027));
#75674=CARTESIAN_POINT('Ctrl Pts',(-19.9762362610291,-17.2377798355797,
-4.82908236895107));
#75675=CARTESIAN_POINT('Ctrl Pts',(-19.973348857078,-17.2356911377957,-4.82929794843881));
#75676=CARTESIAN_POINT('Ctrl Pts',(-19.9670611496364,-17.2311668602427,
-4.8297676626275));
#75677=CARTESIAN_POINT('Ctrl Pts',(-19.9636589425287,-17.2287340953903,
-4.83002197954957));
#75678=CARTESIAN_POINT('Ctrl Pts',(-19.9540764340201,-17.2219249019935,
-4.83073867367661));
#75679=CARTESIAN_POINT('Ctrl Pts',(-19.9478798989552,-17.2175715821844,
-4.8312025854209));
#75680=CARTESIAN_POINT('Ctrl Pts',(-19.9105771489598,-17.1916626868087,
-4.83399740183433));
#75681=CARTESIAN_POINT('Ctrl Pts',(-19.8789228841748,-17.170912573062,-4.83637763839291));
#75682=CARTESIAN_POINT('Ctrl Pts',(-19.772643790887,-17.1052481182388,-4.84435386952129));
#75683=CARTESIAN_POINT('Ctrl Pts',(-19.6958061437537,-17.0640909820055,
-4.85009296043012));
#75684=CARTESIAN_POINT('Ctrl Pts',(-19.4572972918382,-16.9546843936829,
-4.86743040953152));
#75685=CARTESIAN_POINT('Ctrl Pts',(-19.2894390514096,-16.9016489409764,
-4.87894076707727));
#75686=CARTESIAN_POINT('Ctrl Pts',(-19.0943175057405,-16.8657619227104,
-4.89115241284343));
#75687=CARTESIAN_POINT('Ctrl Pts',(-19.0716295238202,-16.8619702417863,
-4.89255651866887));
#75688=CARTESIAN_POINT('Ctrl Pts',(-19.0394420665603,-16.8571288101742,
-4.89452689951001));
#75689=CARTESIAN_POINT('Ctrl Pts',(-19.0299909856626,-16.8557725555024,
-4.89510283244979));
#75690=CARTESIAN_POINT('Ctrl Pts',(-19.0146187594493,-16.8536726380584,
-4.89603541559247));
#75691=CARTESIAN_POINT('Ctrl Pts',(-19.0087031542095,-16.852890001875,-4.89639329396217));
#75692=CARTESIAN_POINT('Ctrl Pts',(-18.9963128079649,-16.8513040303786,
-4.89714081000732));
#75693=CARTESIAN_POINT('Ctrl Pts',(-18.9898374946947,-16.8505055927307,
-4.89753028932198));
#75694=CARTESIAN_POINT('Ctrl Pts',(-18.9744228356038,-16.8486771930396,
-4.89845469933594));
#75695=CARTESIAN_POINT('Ctrl Pts',(-18.9654803640939,-16.8476742611929,
-4.89898877271228));
#75696=CARTESIAN_POINT('Ctrl Pts',(-18.9353259461931,-16.8444868754622,
-4.90078247937644));
#75697=CARTESIAN_POINT('Ctrl Pts',(-18.9140870314545,-16.8425658539026,
-4.90203382867938));
#75698=CARTESIAN_POINT('Ctrl Pts',(-18.7982688068135,-16.8338523528477,
-4.90879743545244));
#75699=CARTESIAN_POINT('Ctrl Pts',(-18.7033386434557,-16.8330986696004,
-4.91411649058406));
#75700=CARTESIAN_POINT('Ctrl Pts',(-18.4394827966976,-16.8487470235508,
-4.92865997844835));
#75701=CARTESIAN_POINT('Ctrl Pts',(-18.2721344894038,-16.8790595276087,
-4.93757834575934));
#75702=CARTESIAN_POINT('Ctrl Pts',(-18.073699387599,-16.9402465966317,-4.94942153759797));
#75703=CARTESIAN_POINT('Ctrl Pts',(-18.0375041290859,-16.9524896227224,
-4.95163836765537));
#75704=CARTESIAN_POINT('Ctrl Pts',(-17.9948815496122,-16.9682043581939,
-4.95433857606212));
#75705=CARTESIAN_POINT('Ctrl Pts',(-17.988113533526,-16.970739136838,-4.95477006902078));
#75706=CARTESIAN_POINT('Ctrl Pts',(-17.9771169276943,-16.974921951183,-4.95547580868114));
#75707=CARTESIAN_POINT('Ctrl Pts',(-17.9728803606414,-16.9765490413683,
-4.95574883248008));
#75708=CARTESIAN_POINT('Ctrl Pts',(-17.9653223641581,-16.9794796773338,
-4.95623798003841));
#75709=CARTESIAN_POINT('Ctrl Pts',(-17.9619989686874,-16.9807780088053,
-4.95645378912896));
#75710=CARTESIAN_POINT('Ctrl Pts',(-17.9548271270823,-16.9836007092489,
-4.95692107648361));
#75711=CARTESIAN_POINT('Ctrl Pts',(-17.9509799189032,-16.9851279437539,
-4.95717272114551));
#75712=CARTESIAN_POINT('Ctrl Pts',(-17.9402910535353,-16.9894074564656,
-4.95787454574103));
#75713=CARTESIAN_POINT('Ctrl Pts',(-17.9334593387876,-16.9921841847513,
-4.95832616167301));
#75714=CARTESIAN_POINT('Ctrl Pts',(-17.8947004582634,-17.0081740781143,
-4.96090514637648));
#75715=CARTESIAN_POINT('Ctrl Pts',(-17.8630880106106,-17.0221308532686,
-4.96307356553371));
#75716=CARTESIAN_POINT('Ctrl Pts',(-17.7641680976425,-17.068728989231,-4.97003473754875));
#75717=CARTESIAN_POINT('Ctrl Pts',(-17.6982440524071,-17.1041656731925,
-4.97493571902539));
#75718=CARTESIAN_POINT('Ctrl Pts',(-17.4686237155528,-17.2437491694053,
-4.99265950552603));
#75719=CARTESIAN_POINT('Ctrl Pts',(-17.3174956185351,-17.3668044597351,
-5.00547447246498));
#75720=CARTESIAN_POINT('Ctrl Pts',(-17.1708087165715,-17.5242152144634,
-5.01869370746706));
#75721=CARTESIAN_POINT('Ctrl Pts',(-17.1566211235977,-17.5399049912863,
-5.01998335157798));
#75722=CARTESIAN_POINT('Ctrl Pts',(-17.137194266815,-17.562046978977,-5.02176547919559));
#75723=CARTESIAN_POINT('Ctrl Pts',(-17.1317546068941,-17.5683209716385,
-5.02226631761537));
#75724=CARTESIAN_POINT('Ctrl Pts',(-17.1224238907934,-17.5792116354617,
-5.02312865197092));
#75725=CARTESIAN_POINT('Ctrl Pts',(-17.1185154401928,-17.5838132116645,
-5.0234908652011));
#75726=CARTESIAN_POINT('Ctrl Pts',(-17.1104578906896,-17.5933823535067,
-5.02423970368474));
#75727=CARTESIAN_POINT('Ctrl Pts',(-17.1063117761606,-17.5983523584487,
-5.02462620429654));
#75728=CARTESIAN_POINT('Ctrl Pts',(-17.0966468974293,-17.6100463926137,
-5.02552998315794));
#75729=CARTESIAN_POINT('Ctrl Pts',(-17.0911466283647,-17.6167856091155,
-5.02604650678409));
#75730=CARTESIAN_POINT('Ctrl Pts',(-17.0733869430483,-17.6388215851803,
-5.0277216343407));
#75731=CARTESIAN_POINT('Ctrl Pts',(-17.0612981949239,-17.6542550391029,
-5.02887339664198));
#75732=CARTESIAN_POINT('Ctrl Pts',(-17.0003521246543,-17.7343303634945,
-5.03474408331668));
#75733=CARTESIAN_POINT('Ctrl Pts',(-16.9550180180235,-17.8015742178492,
-5.03932427760283));
#75734=CARTESIAN_POINT('Ctrl Pts',(-16.8275649624743,-18.0162503607255,
-5.05316172570832));
#75735=CARTESIAN_POINT('Ctrl Pts',(-16.7591218671788,-18.170993865104,-5.06203404371519));
#75736=CARTESIAN_POINT('Ctrl Pts',(-16.6939626106512,-18.3838024684258,
-5.07454412732924));
#75737=CARTESIAN_POINT('Ctrl Pts',(-16.6801439271473,-18.4359814291646,
-5.0776392203901));
#75738=CARTESIAN_POINT('Ctrl Pts',(-16.6664208298208,-18.4971573698522,
-5.08135962970058));
#75739=CARTESIAN_POINT('Ctrl Pts',(-16.6645600091364,-18.505700144063,-5.08188121416451));
#75740=CARTESIAN_POINT('Ctrl Pts',(-16.6618241473143,-18.518645204009,-5.08267502688484));
#75741=CARTESIAN_POINT('Ctrl Pts',(-16.6609100756644,-18.5230392693642,
-5.08294507726038));
#75742=CARTESIAN_POINT('Ctrl Pts',(-16.659295173072,-18.5309280520047,-5.08343103368197));
#75743=CARTESIAN_POINT('Ctrl Pts',(-16.658589189201,-18.5344216595742,-5.08364664197009));
#75744=CARTESIAN_POINT('Ctrl Pts',(-16.6570751835372,-18.542012504429,-5.08411598915867));
#75745=CARTESIAN_POINT('Ctrl Pts',(-16.6562704721389,-18.5461103005463,
-5.08436990793588));
#75746=CARTESIAN_POINT('Ctrl Pts',(-16.6540462440104,-18.5576165899978,
-5.08508438019229));
#75747=CARTESIAN_POINT('Ctrl Pts',(-16.6526542085713,-18.5650302418684,
-5.08554645329898));
#75748=CARTESIAN_POINT('Ctrl Pts',(-16.6446091918002,-18.6091756448927,
-5.08830755001023));
#75749=CARTESIAN_POINT('Ctrl Pts',(-16.6388895262453,-18.6460683158044,
-5.09065455983395));
#75750=CARTESIAN_POINT('Ctrl Pts',(-16.6233425450778,-18.7674708982687,
-5.09846553204106));
#75751=CARTESIAN_POINT('Ctrl Pts',(-16.6176332923926,-18.8524210077317,
-5.10406664451242));
#75752=CARTESIAN_POINT('Ctrl Pts',(-16.6158271713325,-19.115707342499,-5.12145998327809));
#75753=CARTESIAN_POINT('Ctrl Pts',(-16.6371175926894,-19.2934160825607,
-5.13317340558461));
#75754=CARTESIAN_POINT('Ctrl Pts',(-16.6859740385284,-19.4884674680425,
-5.14554744331572));
#75755=CARTESIAN_POINT('Ctrl Pts',(-16.6918639708136,-19.5104695023179,
-5.14693756203306));
#75756=CARTESIAN_POINT('Ctrl Pts',(-16.7007152895663,-19.5415190724221,
-5.14889189946053));
#75757=CARTESIAN_POINT('Ctrl Pts',(-16.7033842292597,-19.5506476815881,
-5.14946556413045));
#75758=CARTESIAN_POINT('Ctrl Pts',(-16.7078257583753,-19.5654675773988,
-5.15039547802102));
#75759=CARTESIAN_POINT('Ctrl Pts',(-16.7095610053027,-19.5711698343924,
-5.15075294151145));
#75760=CARTESIAN_POINT('Ctrl Pts',(-16.7132478150417,-19.5831039934743,
-5.15150038777389));
#75761=CARTESIAN_POINT('Ctrl Pts',(-16.715204179666,-19.5893343556317,-5.15189020868588));
#75762=CARTESIAN_POINT('Ctrl Pts',(-16.7199347134666,-19.6041591673668,
-5.15281688090697));
#75763=CARTESIAN_POINT('Ctrl Pts',(-16.7227351250823,-19.6127451587187,
-5.15335286356986));
#75764=CARTESIAN_POINT('Ctrl Pts',(-16.7323932945808,-19.6417264545518,
-5.15515982128339));
#75765=CARTESIAN_POINT('Ctrl Pts',(-16.7395071627998,-19.6620354624039,
-5.1564223419963));
#75766=CARTESIAN_POINT('Ctrl Pts',(-16.8091034175928,-19.8514169975164,
-5.16816955223975));
#75767=CARTESIAN_POINT('Ctrl Pts',(-16.8926263182991,-20.0119658805139,
-5.17784950510681));
#75768=CARTESIAN_POINT('Ctrl Pts',(-17.0637496983472,-20.2582400141959,
-5.19417301241013));
#75769=CARTESIAN_POINT('Ctrl Pts',(-17.1402042650119,-20.3505012982325,
-5.20073948503146));
#75770=CARTESIAN_POINT('Ctrl Pts',(-17.2307011257851,-20.4425945916122,
-5.20839126428913));
#75771=CARTESIAN_POINT('Ctrl Pts',(-17.2374234109787,-20.4493437305056,
-5.20895904648627));
#75772=CARTESIAN_POINT('Ctrl Pts',(-17.247449426917,-20.4592748355662,-5.20980540341093));
#75773=CARTESIAN_POINT('Ctrl Pts',(-17.2507184263142,-20.4624919094522,
-5.21008128688877));
#75774=CARTESIAN_POINT('Ctrl Pts',(-17.256552161142,-20.468195780738,-5.21057354661375));
#75775=CARTESIAN_POINT('Ctrl Pts',(-17.2591127623494,-20.4706867346699,
-5.21078959197053));
#75776=CARTESIAN_POINT('Ctrl Pts',(-17.2646303350937,-20.476027115976,-5.21125509407607));
#75777=CARTESIAN_POINT('Ctrl Pts',(-17.2675892522231,-20.4788743826915,
-5.21150470502881));
#75778=CARTESIAN_POINT('Ctrl Pts',(-17.2757767494028,-20.4867071855417,
-5.2121952769454));
#75779=CARTESIAN_POINT('Ctrl Pts',(-17.281022537944,-20.4916745387342,-5.21263760128345));
#75780=CARTESIAN_POINT('Ctrl Pts',(-17.3098521404919,-20.51869538535,-5.21506728156679));
#75781=CARTESIAN_POINT('Ctrl Pts',(-17.3339113496193,-20.5402326856838,
-5.21709041868506));
#75782=CARTESIAN_POINT('Ctrl Pts',(-17.4822884581557,-20.6670650010254,
-5.22949111444313));
#75783=CARTESIAN_POINT('Ctrl Pts',(-17.6179259216366,-20.7582691633827,
-5.24046260206151));
#75784=CARTESIAN_POINT('Ctrl Pts',(-17.8665680921382,-20.8866632224974,
-5.25874172871462));
#75785=CARTESIAN_POINT('Ctrl Pts',(-17.9747357728673,-20.9316175290176,
-5.26618974429921));
#75786=CARTESIAN_POINT('Ctrl Pts',(-18.0996602058279,-20.9717785821859,
-5.27420185751572));
#75787=CARTESIAN_POINT('Ctrl Pts',(-18.1132848903825,-20.9760072292008,
-5.275068346271));
#75788=CARTESIAN_POINT('Ctrl Pts',(-18.1350443039693,-20.9825202374226,
-5.27644075236257));
#75789=CARTESIAN_POINT('Ctrl Pts',(-18.1431515801917,-20.9848941213038,
-5.27694958516799));
#75790=CARTESIAN_POINT('Ctrl Pts',(-18.1574791314231,-20.9889964070899,
-5.27784446579406));
#75791=CARTESIAN_POINT('Ctrl Pts',(-18.1636934695377,-20.9907449907101,
-5.27823116744733));
#75792=CARTESIAN_POINT('Ctrl Pts',(-18.1765671885943,-20.9943039155187,
-5.279029331701));
#75793=CARTESIAN_POINT('Ctrl Pts',(-18.1832276252643,-20.9961101769564,
-5.27944065771707));
#75794=CARTESIAN_POINT('Ctrl Pts',(-18.2003549537786,-21.0006651929261,
-5.28049429900883));
#75795=CARTESIAN_POINT('Ctrl Pts',(-18.2108343871675,-21.0033663388569,
-5.28113506762424));
#75796=CARTESIAN_POINT('Ctrl Pts',(-18.2547281810703,-21.0143220291703,
-5.2838031282882));
#75797=CARTESIAN_POINT('Ctrl Pts',(-18.2883217226217,-21.0218417089202,
-5.28580672432724));
#75798=CARTESIAN_POINT('Ctrl Pts',(-18.3763829169174,-21.0393100580302,
-5.29097124066264));
#75799=CARTESIAN_POINT('Ctrl Pts',(-18.4310846950575,-21.0479475726715,
-5.29409236020354));
#75800=CARTESIAN_POINT('Ctrl Pts',(-18.594865672738,-21.0672618694223,-5.30326042037942));
#75801=CARTESIAN_POINT('Ctrl Pts',(-18.7045007947106,-21.0716277488065,
-5.30915871255457));
#75802=CARTESIAN_POINT('Ctrl Pts',(-18.8739982842528,-21.0652195180955,
-5.31839460246183));
#75803=CARTESIAN_POINT('Ctrl Pts',(-18.9338894852895,-21.0603974491121,
-5.32168325163462));
#75804=CARTESIAN_POINT('Ctrl Pts',(-19.051583025937,-21.0458615288197,-5.32832474052661));
#75805=CARTESIAN_POINT('Ctrl Pts',(-19.1093464228304,-21.0362813711832,
-5.3316711224459));
#75806=CARTESIAN_POINT('Ctrl Pts',(-19.1753598861204,-21.0224999228472,
-5.3356714603907));
#75807=CARTESIAN_POINT('Ctrl Pts',(-19.1840751004848,-21.0206229422488,
-5.33620317116771));
#75808=CARTESIAN_POINT('Ctrl Pts',(-19.1971954794535,-21.0177103919284,
-5.33700939648203));
#75809=CARTESIAN_POINT('Ctrl Pts',(-19.2016097308295,-21.0167156255202,
-5.33728163019653));
#75810=CARTESIAN_POINT('Ctrl Pts',(-19.2094979154796,-21.0149114028133,
-5.33776992516007));
#75811=CARTESIAN_POINT('Ctrl Pts',(-19.2129730221529,-21.0141073122575,
-5.33798567622846));
#75812=CARTESIAN_POINT('Ctrl Pts',(-19.2204857561669,-21.0123489562675,
-5.33845348976367));
#75813=CARTESIAN_POINT('Ctrl Pts',(-19.2245225594754,-21.0113916165969,
-5.33870572212657));
#75814=CARTESIAN_POINT('Ctrl Pts',(-19.2357692537056,-21.0086894863316,
-5.33941080843201));
#75815=CARTESIAN_POINT('Ctrl Pts',(-19.2429727446804,-21.006918676877,-5.33986511973635));
#75816=CARTESIAN_POINT('Ctrl Pts',(-19.2843476322461,-20.9965167322221,
-5.34248954072507));
#75817=CARTESIAN_POINT('Ctrl Pts',(-19.3183064302945,-20.9870717047429,
-5.34470237886729));
#75818=CARTESIAN_POINT('Ctrl Pts',(-19.4259113774478,-20.9542281709081,
-5.351869160434));
#75819=CARTESIAN_POINT('Ctrl Pts',(-19.4985163961957,-20.927644720345,-5.35693806707062));
#75820=CARTESIAN_POINT('Ctrl Pts',(-19.7398391010537,-20.8239896048735,
-5.37426982775066));
#75821=CARTESIAN_POINT('Ctrl Pts',(-19.8998680925405,-20.7287486842645,
-5.38651055335972));
#75822=CARTESIAN_POINT('Ctrl Pts',(-20.0650216354066,-20.5984178310324,
-5.39948466512282));
#75823=CARTESIAN_POINT('Ctrl Pts',(-20.0843145167135,-20.5826321036715,
-5.40100815747494));
#75824=CARTESIAN_POINT('Ctrl Pts',(-20.1108536419003,-20.5601232872844,
-5.40311585822893));
#75825=CARTESIAN_POINT('Ctrl Pts',(-20.1183378379905,-20.5536851169297,
-5.40371161556621));
#75826=CARTESIAN_POINT('Ctrl Pts',(-20.1303182962737,-20.5432323968035,
-5.40466759882434));
#75827=CARTESIAN_POINT('Ctrl Pts',(-20.1348428614278,-20.5392506430618,
-5.40502917650968));
#75828=CARTESIAN_POINT('Ctrl Pts',(-20.1439056124033,-20.5312062129399,
-5.40575453771887));
#75829=CARTESIAN_POINT('Ctrl Pts',(-20.1484433925525,-20.527143164711,-5.40611830063494));
#75830=CARTESIAN_POINT('Ctrl Pts',(-20.1591474237462,-20.517475408303,-5.40697776366185));
#75831=CARTESIAN_POINT('Ctrl Pts',(-20.1652982732665,-20.5118537397415,
-5.40747274187518));
#75832=CARTESIAN_POINT('Ctrl Pts',(-20.1844111719896,-20.4941769562572,
-5.40901443777274));
#75833=CARTESIAN_POINT('Ctrl Pts',(-20.1972555320385,-20.481995296866,-5.41005574820745));
#75834=CARTESIAN_POINT('Ctrl Pts',(-20.2267942716557,-20.4532683338876,
-5.41246410561028));
#75835=CARTESIAN_POINT('Ctrl Pts',(-20.243369074385,-20.4366031143289,-5.41382590490901));
#75836=CARTESIAN_POINT('Ctrl Pts',(-20.2996028027923,-20.3781471656349,
-5.41848799285678));
#75837=CARTESIAN_POINT('Ctrl Pts',(-20.3378326805298,-20.3350145802317,
-5.42173082938301));
#75838=CARTESIAN_POINT('Ctrl Pts',(-20.4753967613963,-20.1664214927511,
-5.43380595582215));
#75839=CARTESIAN_POINT('Ctrl Pts',(-20.5621526223952,-20.0314143648029,
-5.44225421016962));
#75840=CARTESIAN_POINT('Ctrl Pts',(-20.6392394613238,-19.8750162295932,
-5.45197646644191));
#75841=CARTESIAN_POINT('Ctrl Pts',(-20.6454737662907,-19.8620353795311,
-5.45278327657294));
#75842=CARTESIAN_POINT('Ctrl Pts',(-20.6532775002094,-19.8453526858455,
-5.45382122623665));
#75843=CARTESIAN_POINT('Ctrl Pts',(-20.6549695786014,-19.8417083914765,
-5.45404802790572));
#75844=CARTESIAN_POINT('Ctrl Pts',(-20.6763865889926,-19.7952358347431,
-5.45694131536283));
#75845=CARTESIAN_POINT('Ctrl Pts',(-20.6946840974345,-19.7517683888456,
-5.45965908549561));
#75846=CARTESIAN_POINT('Ctrl Pts',(-20.7142605909899,-19.7005427147481,
-5.46291526173001));
#75847=CARTESIAN_POINT('Ctrl Pts',(-20.7169681034621,-19.6933404754991,
-5.46337428170636));
#75848=CARTESIAN_POINT('Ctrl Pts',(-20.7206230839558,-19.6834545923031,
-5.464006196137));
#75849=CARTESIAN_POINT('Ctrl Pts',(-20.7216045310241,-19.6807834564002,
-5.46417712267594));
#75850=CARTESIAN_POINT('Ctrl Pts',(-20.7225805821191,-19.6781103693095,
-5.46434836675477));
#75851=CARTESIAN_POINT('Ctrl Pts',(-20.7225806512393,-19.6781101800116,
-5.24452704027197));
#75852=CARTESIAN_POINT('Ctrl Pts',(-20.701412508508,-19.7360828682028,-5.24117482982837));
#75853=CARTESIAN_POINT('Ctrl Pts',(-20.6777012517521,-19.7931519033798,
-5.23782819558385));
#75854=CARTESIAN_POINT('Ctrl Pts',(-20.6249328031585,-19.9059353994099,
-5.23098485563475));
#75855=CARTESIAN_POINT('Ctrl Pts',(-20.5958562751286,-19.9615096209843,
-5.22749301409946));
#75856=CARTESIAN_POINT('Ctrl Pts',(-20.5488219989097,-20.0424431755143,
-5.22210866281003));
#75857=CARTESIAN_POINT('Ctrl Pts',(-20.5327016317153,-20.0688336580986,
-5.2203028599762));
#75858=CARTESIAN_POINT('Ctrl Pts',(-20.5121619813386,-20.1008602082743,
-5.21803693468279));
#75859=CARTESIAN_POINT('Ctrl Pts',(-20.5082836583955,-20.1068408142658,
-5.21761053618827));
#75860=CARTESIAN_POINT('Ctrl Pts',(-20.5021352896038,-20.1162178859737,
-5.21693664317567));
#75861=CARTESIAN_POINT('Ctrl Pts',(-20.4998854482371,-20.1196276253236,
-5.21669048061429));
#75862=CARTESIAN_POINT('Ctrl Pts',(-20.4956478281365,-20.126009674404,-5.21622759205944));
#75863=CARTESIAN_POINT('Ctrl Pts',(-20.4936623833027,-20.1289834672085,
-5.21601102225427));
#75864=CARTESIAN_POINT('Ctrl Pts',(-20.489094629283,-20.135787642446,-5.2155134878238));
#75865=CARTESIAN_POINT('Ctrl Pts',(-20.4865073176134,-20.1396146011748,
-5.21523218831693));
#75866=CARTESIAN_POINT('Ctrl Pts',(-20.4784512074551,-20.1514469472664,
-5.21435798358808));
#75867=CARTESIAN_POINT('Ctrl Pts',(-20.4729400168071,-20.1594231256028,
-5.21376231253154));
#75868=CARTESIAN_POINT('Ctrl Pts',(-20.4106714931198,-20.2482318523178,
-5.20706093232178));
#75869=CARTESIAN_POINT('Ctrl Pts',(-20.348384924969,-20.325026218361,-5.20062766912869));
#75870=CARTESIAN_POINT('Ctrl Pts',(-20.166459304275,-20.5197658532761,-5.18307321918491));
#75871=CARTESIAN_POINT('Ctrl Pts',(-20.0377573524291,-20.6283241657014,
-5.17192751593069));
#75872=CARTESIAN_POINT('Ctrl Pts',(-19.871209325056,-20.7379003579268,-5.15940136273166));
#75873=CARTESIAN_POINT('Ctrl Pts',(-19.8444569005771,-20.7546565880787,
-5.1574387430459));
#75874=CARTESIAN_POINT('Ctrl Pts',(-19.8041717030768,-20.7786516911934,
-5.15455521984329));
#75875=CARTESIAN_POINT('Ctrl Pts',(-19.7909197325146,-20.7863512677238,
-5.15361791191717));
#75876=CARTESIAN_POINT('Ctrl Pts',(-19.766647314889,-20.8001035037864,-5.15192121243094));
#75877=CARTESIAN_POINT('Ctrl Pts',(-19.7556544276193,-20.8062031385127,
-5.15116015889834));
#75878=CARTESIAN_POINT('Ctrl Pts',(-19.7382624440951,-20.8156518152792,
-5.14996747465325));
#75879=CARTESIAN_POINT('Ctrl Pts',(-19.731899561837,-20.8190665793456,-5.14953350372701));
#75880=CARTESIAN_POINT('Ctrl Pts',(-19.7254731395678,-20.8224732065016,
-5.14909755972947));
#75881=CARTESIAN_POINT('Ctrl Pts',(-19.7254270075463,-20.8224976587616,
-5.14909443043108));
#75882=CARTESIAN_POINT('Ctrl Pts',(-19.7253331174823,-20.8225474207042,
-5.14908806178418));
#75883=CARTESIAN_POINT('Ctrl Pts',(-19.7252853582169,-20.8225727308782,
-5.14908482236145));
#75884=CARTESIAN_POINT('Ctrl Pts',(-19.725188154278,-20.8226242396454,-5.14907822946432));
#75885=CARTESIAN_POINT('Ctrl Pts',(-19.7251387087258,-20.8226504385362,
-5.14907487593968));
#75886=CARTESIAN_POINT('Ctrl Pts',(-19.7250380707156,-20.8227037568112,
-5.1490680506963));
#75887=CARTESIAN_POINT('Ctrl Pts',(-19.7249868772868,-20.8227308765295,
-5.14906457892176));
#75888=CARTESIAN_POINT('Ctrl Pts',(-19.7248826796944,-20.8227860697253,
-5.14905751288047));
#75889=CARTESIAN_POINT('Ctrl Pts',(-19.7248296747771,-20.8228141434087,
-5.14905391857337));
#75890=CARTESIAN_POINT('Ctrl Pts',(-19.7247217880893,-20.8228712789663,
-5.14904660301622));
#75891=CARTESIAN_POINT('Ctrl Pts',(-19.7246669055455,-20.8229003410425,
-5.1490428817253));
#75892=CARTESIAN_POINT('Ctrl Pts',(-19.7245551950909,-20.8229594890356,
-5.1490353075901));
#75893=CARTESIAN_POINT('Ctrl Pts',(-19.7244983664698,-20.8229895751058,
-5.14903145471009));
#75894=CARTESIAN_POINT('Ctrl Pts',(-19.724382693013,-20.8230508079185,-5.14902361263113));
#75895=CARTESIAN_POINT('Ctrl Pts',(-19.7243238472484,-20.8230819549137,
-5.14901962338252));
#75896=CARTESIAN_POINT('Ctrl Pts',(-19.7242040658153,-20.8231453478539,
-5.14901150361136));
#75897=CARTESIAN_POINT('Ctrl Pts',(-19.7241431295488,-20.823177593859,-5.14900737306257));
#75898=CARTESIAN_POINT('Ctrl Pts',(-19.7240190907779,-20.8232432244343,
-5.1489989655602));
#75899=CARTESIAN_POINT('Ctrl Pts',(-19.7239559877364,-20.8232766090135,
-5.14899468858556));
#75900=CARTESIAN_POINT('Ctrl Pts',(-19.7238275365145,-20.8233445576436,
-5.14898598293039));
#75901=CARTESIAN_POINT('Ctrl Pts',(-19.7237621877721,-20.8233791216965,
-5.14898155422824));
#75902=CARTESIAN_POINT('Ctrl Pts',(-19.7236291613103,-20.8234494727203,
-5.14897253948635));
#75903=CARTESIAN_POINT('Ctrl Pts',(-19.7235614862716,-20.8234852579563,
-5.14896795364603));
#75904=CARTESIAN_POINT('Ctrl Pts',(-19.7234348771654,-20.8235521975867,
-5.14895937476716));
#75905=CARTESIAN_POINT('Ctrl Pts',(-19.7233759422767,-20.8235833535505,
-5.14895538160964));
#75906=CARTESIAN_POINT('Ctrl Pts',(-19.72324832144,-20.8236508126687,-5.14894673503811));
#75907=CARTESIAN_POINT('Ctrl Pts',(-19.7231796338908,-20.8236871153938,
-5.14894208158675));
#75908=CARTESIAN_POINT('Ctrl Pts',(-19.7230309113934,-20.8237657076947,
-5.14893200650377));
#75909=CARTESIAN_POINT('Ctrl Pts',(-19.72295087472,-20.8238079964528,-5.14892658485174));
#75910=CARTESIAN_POINT('Ctrl Pts',(-19.7227776039674,-20.8238995328303,
-5.14891484835399));
#75911=CARTESIAN_POINT('Ctrl Pts',(-19.7226843682897,-20.8239487789514,
-5.14890853353066));
#75912=CARTESIAN_POINT('Ctrl Pts',(-19.7224825594817,-20.8240553529944,
-5.14889486615894));
#75913=CARTESIAN_POINT('Ctrl Pts',(-19.7223739845068,-20.8241126787202,
-5.14888751366245));
#75914=CARTESIAN_POINT('Ctrl Pts',(-19.7221390264431,-20.8242367064135,
-5.14887160419482));
#75915=CARTESIAN_POINT('Ctrl Pts',(-19.7220126419178,-20.8243034048552,
-5.14886304736537));
#75916=CARTESIAN_POINT('Ctrl Pts',(-19.7217267158614,-20.8244542630756,
-5.14884369088451));
#75917=CARTESIAN_POINT('Ctrl Pts',(-19.7215671702725,-20.8245384152899,
-5.14883289149962));
#75918=CARTESIAN_POINT('Ctrl Pts',(-19.7156957099711,-20.8276343539857,
-5.14843551524378));
#75919=CARTESIAN_POINT('Ctrl Pts',(-19.709970007852,-20.8306200366296,-5.14804986596609));
#75920=CARTESIAN_POINT('Ctrl Pts',(-19.6967131593703,-20.8374558897946,
-5.14716120869103));
#75921=CARTESIAN_POINT('Ctrl Pts',(-19.6891723883767,-20.8412872336508,
-5.14665886789929));
#75922=CARTESIAN_POINT('Ctrl Pts',(-19.6688197918885,-20.8514750582571,
-5.14531135253574));
#75923=CARTESIAN_POINT('Ctrl Pts',(-19.6559660407866,-20.8577471434665,
-5.14446912563664));
#75924=CARTESIAN_POINT('Ctrl Pts',(-19.5375051525996,-20.9140719774847,
-5.13678489397074));
#75925=CARTESIAN_POINT('Ctrl Pts',(-19.4279803503686,-20.9554329321603,
-5.13025973450201));
#75926=CARTESIAN_POINT('Ctrl Pts',(-19.1589144830927,-21.0323093763631,
-5.11494068576974));
#75927=CARTESIAN_POINT('Ctrl Pts',(-18.9976163601083,-21.0588302951818,
-5.10633050195121));
#75928=CARTESIAN_POINT('Ctrl Pts',(-18.802657888277,-21.0681324864585,-5.09512065436378));
#75929=CARTESIAN_POINT('Ctrl Pts',(-18.7703916462459,-21.0689331585919,
-5.09323794340659));
#75930=CARTESIAN_POINT('Ctrl Pts',(-18.7308982435761,-21.069010051562,-5.09088638021151));
#75931=CARTESIAN_POINT('Ctrl Pts',(-18.7236748263827,-21.0689871437202,
-5.09045434401347));
#75932=CARTESIAN_POINT('Ctrl Pts',(-18.7123457678714,-21.0688932317858,
-5.08977352241842));
#75933=CARTESIAN_POINT('Ctrl Pts',(-18.7082398968279,-21.0688472493251,
-5.08952611497209));
#75934=CARTESIAN_POINT('Ctrl Pts',(-18.7005621239105,-21.0687389236498,
-5.08906218984495));
#75935=CARTESIAN_POINT('Ctrl Pts',(-18.6969902372455,-21.0686794842991,
-5.08884583621685));
#75936=CARTESIAN_POINT('Ctrl Pts',(-18.6888325025982,-21.068523077253,-5.08835052346686));
#75937=CARTESIAN_POINT('Ctrl Pts',(-18.684246824114,-21.0684202465344,-5.08807124063714));
#75938=CARTESIAN_POINT('Ctrl Pts',(-18.6701371321334,-21.068057964413,-5.08720936039492));
#75939=CARTESIAN_POINT('Ctrl Pts',(-18.6606146606291,-21.0677491247349,
-5.08662410618977));
#75940=CARTESIAN_POINT('Ctrl Pts',(-18.5315868426045,-21.0626923044512,
-5.07864842441961));
#75941=CARTESIAN_POINT('Ctrl Pts',(-18.4127041625726,-21.0478901317207,
-5.07078117013936));
#75942=CARTESIAN_POINT('Ctrl Pts',(-18.1891105519226,-21.0005750194232,
-5.05568285004451));
#75943=CARTESIAN_POINT('Ctrl Pts',(-18.0843911619887,-20.9698146482621,
-5.04847967986346));
#75944=CARTESIAN_POINT('Ctrl Pts',(-17.9123447350746,-20.9044863820415,
-5.03665529331572));
#75945=CARTESIAN_POINT('Ctrl Pts',(-17.8436493653112,-20.8741337988686,
-5.03193390296942));
#75946=CARTESIAN_POINT('Ctrl Pts',(-17.7599283654259,-20.8316880653889,
-5.02618361841979));
#75947=CARTESIAN_POINT('Ctrl Pts',(-17.743266084539,-20.8229594108491,-5.02503920847367));
#75948=CARTESIAN_POINT('Ctrl Pts',(-17.7191977435569,-20.8099393318205,
-5.02338571958801));
#75949=CARTESIAN_POINT('Ctrl Pts',(-17.7116982316541,-20.8058234215264,
-5.02287044425809));
#75950=CARTESIAN_POINT('Ctrl Pts',(-17.698588966041,-20.7985250021227,-5.02196956096895));
#75951=CARTESIAN_POINT('Ctrl Pts',(-17.6929684619539,-20.7953621269109,
-5.02158325704022));
#75952=CARTESIAN_POINT('Ctrl Pts',(-17.6820796660661,-20.7891688945382,
-5.0208347107161));
#75953=CARTESIAN_POINT('Ctrl Pts',(-17.676809803319,-20.7861414409006,-5.02047236877512));
#75954=CARTESIAN_POINT('Ctrl Pts',(-17.6642380443395,-20.778846978069,-5.01960776566425));
#75955=CARTESIAN_POINT('Ctrl Pts',(-17.6569485004485,-20.7745588038596,
-5.01910627497618));
#75956=CARTESIAN_POINT('Ctrl Pts',(-17.6307077474832,-20.7589099063787,
-5.01730024107344));
#75957=CARTESIAN_POINT('Ctrl Pts',(-17.6119085675366,-20.7472960969243,
-5.01600492121));
#75958=CARTESIAN_POINT('Ctrl Pts',(-17.4368585585138,-20.6353292242278,
-5.00391935116773));
#75959=CARTESIAN_POINT('Ctrl Pts',(-17.2942716497095,-20.5151255478294,
-4.99398693202737));
#75960=CARTESIAN_POINT('Ctrl Pts',(-17.1152599276401,-20.3186676595058,
-4.97949760014236));
#75961=CARTESIAN_POINT('Ctrl Pts',(-17.0647371429149,-20.2564766861742,
-4.97509416313345));
#75962=CARTESIAN_POINT('Ctrl Pts',(-16.996776374576,-20.1623882895478,-4.96845494489296));
#75963=CARTESIAN_POINT('Ctrl Pts',(-16.9764407449288,-20.1326654280783,
-4.96636033250357));
#75964=CARTESIAN_POINT('Ctrl Pts',(-16.9528176247318,-20.096173969665,-4.9637733559986));
#75965=CARTESIAN_POINT('Ctrl Pts',(-16.9487941436464,-20.0898860986497,
-4.96332705308486));
#75966=CARTESIAN_POINT('Ctrl Pts',(-16.9425809731613,-20.0800621295238,
-4.96262871174907));
#75967=CARTESIAN_POINT('Ctrl Pts',(-16.9403682606245,-20.0765405642337,
-4.96237817067017));
#75968=CARTESIAN_POINT('Ctrl Pts',(-16.9362776969439,-20.0699875835524,
-4.96191152822627));
#75969=CARTESIAN_POINT('Ctrl Pts',(-16.9343971224923,-20.0669579357728,
-4.96169561035057));
#75970=CARTESIAN_POINT('Ctrl Pts',(-16.9301549244374,-20.0600849658929,
-4.96120539646741));
#75971=CARTESIAN_POINT('Ctrl Pts',(-16.9277979369043,-20.0562388576151,
-4.96093080280682));
#75972=CARTESIAN_POINT('Ctrl Pts',(-16.9217435016202,-20.0462880438659,
-4.96021972596023));
#75973=CARTESIAN_POINT('Ctrl Pts',(-16.9180646357774,-20.0401721777926,
-4.95978207540537));
#75974=CARTESIAN_POINT('Ctrl Pts',(-16.8956520622646,-20.0024826101223,
-4.95708180604267));
#75975=CARTESIAN_POINT('Ctrl Pts',(-16.8777125917328,-19.9704466296272,
-4.95477288084186));
#75976=CARTESIAN_POINT('Ctrl Pts',(-16.7812823468265,-19.7872238540327,
-4.94155895734582));
#75977=CARTESIAN_POINT('Ctrl Pts',(-16.7204314381137,-19.627462679868,-4.930065518428));
#75978=CARTESIAN_POINT('Ctrl Pts',(-16.6563720880417,-19.3694561012144,
-4.91278860405544));
#75979=CARTESIAN_POINT('Ctrl Pts',(-16.6396562380864,-19.2753199787532,
-4.9067213552348));
#75980=CARTESIAN_POINT('Ctrl Pts',(-16.6270442302635,-19.1590857808435,
-4.89953960663383));
#75981=CARTESIAN_POINT('Ctrl Pts',(-16.6250581125698,-19.1377721844143,
-4.89823493270904));
#75982=CARTESIAN_POINT('Ctrl Pts',(-16.6226955445641,-19.1074468109817,
-4.89639537240257));
#75983=CARTESIAN_POINT('Ctrl Pts',(-16.6220529413086,-19.0984576382393,
-4.89585216655937));
#75984=CARTESIAN_POINT('Ctrl Pts',(-16.6210439463346,-19.0829515692758,
-4.89491866842861));
#75985=CARTESIAN_POINT('Ctrl Pts',(-16.6206502597991,-19.0764366316263,
-4.89452752450061));
#75986=CARTESIAN_POINT('Ctrl Pts',(-16.6199544872604,-19.0639649164083,
-4.89378075649995));
#75987=CARTESIAN_POINT('Ctrl Pts',(-16.6196474338811,-19.0580084888501,
-4.89342498024006));
#75988=CARTESIAN_POINT('Ctrl Pts',(-16.6189150599378,-19.0425293199526,
-4.89250264727081));
#75989=CARTESIAN_POINT('Ctrl Pts',(-16.6185288729768,-19.0330047942884,
-4.89193732122574));
#75990=CARTESIAN_POINT('Ctrl Pts',(-16.6174336357373,-19.0005850339198,
-4.89002027993911));
#75991=CARTESIAN_POINT('Ctrl Pts',(-16.6170318259038,-18.9776805368961,
-4.88867817331972));
#75992=CARTESIAN_POINT('Ctrl Pts',(-16.6167704492709,-18.7781623171578,
-4.87708348006839));
#75993=CARTESIAN_POINT('Ctrl Pts',(-16.6386383823485,-18.6022188590461,
-4.86759312005003));
#75994=CARTESIAN_POINT('Ctrl Pts',(-16.7033225289012,-18.347458107908,-4.85328889686386));
#75995=CARTESIAN_POINT('Ctrl Pts',(-16.7296224565645,-18.2652757430582,
-4.84856665876379));
#75996=CARTESIAN_POINT('Ctrl Pts',(-16.7744881232805,-18.1498668095713,
-4.84149558513031));
#75997=CARTESIAN_POINT('Ctrl Pts',(-16.7890515430464,-18.1151729230826,
-4.83930986967051));
#75998=CARTESIAN_POINT('Ctrl Pts',(-16.8076413505476,-18.0739974314149,
-4.83662186527621));
#75999=CARTESIAN_POINT('Ctrl Pts',(-16.8107890926625,-18.0671237607708,
-4.83616994232323));
#76000=CARTESIAN_POINT('Ctrl Pts',(-16.8157341543096,-18.0564763455102,
-4.83546470562457));
#76001=CARTESIAN_POINT('Ctrl Pts',(-16.8175059832761,-18.0526907352522,
-4.83521293744017));
#76002=CARTESIAN_POINT('Ctrl Pts',(-16.8208093575034,-18.0456869925087,
-4.83474519286304));
#76003=CARTESIAN_POINT('Ctrl Pts',(-16.8223378226635,-18.0424674710373,
-4.83452940744883));
#76004=CARTESIAN_POINT('Ctrl Pts',(-16.8258074206715,-18.035206576849,-4.83404101685401));
#76005=CARTESIAN_POINT('Ctrl Pts',(-16.8277532550989,-18.0311675248798,
-4.8337681235017));
#76006=CARTESIAN_POINT('Ctrl Pts',(-16.8335218058151,-18.0192901380843,
-4.83296212984865));
#76007=CARTESIAN_POINT('Ctrl Pts',(-16.8373800891638,-18.0114693195347,
-4.83242689242618));
#76008=CARTESIAN_POINT('Ctrl Pts',(-16.8651908063611,-17.9559634612137,
-4.82859712169009));
#76009=CARTESIAN_POINT('Ctrl Pts',(-16.8908883822631,-17.9091792501178,
-4.82520546127254));
#76010=CARTESIAN_POINT('Ctrl Pts',(-16.9273695634691,-17.848331125134,-4.82062021747684));
#76011=CARTESIAN_POINT('Ctrl Pts',(-16.9366036937779,-17.8333557251065,
-4.8194771529287));
#76012=CARTESIAN_POINT('Ctrl Pts',(-16.9719946087679,-17.7775304117428,
-4.81516520472423));
#76013=CARTESIAN_POINT('Ctrl Pts',(-16.9993656811007,-17.7374690806475,
-4.81196755704903));
#76014=CARTESIAN_POINT('Ctrl Pts',(-17.0928605310547,-17.6102418812309,
-4.80153803629925));
#76015=CARTESIAN_POINT('Ctrl Pts',(-17.1643723371996,-17.5272452590906,
-4.79430523469923));
#76016=CARTESIAN_POINT('Ctrl Pts',(-17.2810731876476,-17.4113089686908,
-4.78373158107755));
#76017=CARTESIAN_POINT('Ctrl Pts',(-17.321667310296,-17.3740131905885,-4.78024235191638));
#76018=CARTESIAN_POINT('Ctrl Pts',(-17.3898211268824,-17.3161366480742,
-4.77468465258231));
#76019=CARTESIAN_POINT('Ctrl Pts',(-17.4165057341725,-17.2945698129473,
-4.77257774142542));
#76020=CARTESIAN_POINT('Ctrl Pts',(-17.4522728780004,-17.2670722838763,
-4.7698411632716));
#76021=CARTESIAN_POINT('Ctrl Pts',(-17.4608922195501,-17.2605502047134,
-4.76918815389577));
#76022=CARTESIAN_POINT('Ctrl Pts',(-17.4750937108824,-17.2499742839813,
-4.76812264827348));
#76023=CARTESIAN_POINT('Ctrl Pts',(-17.4806463157958,-17.2458812682546,
-4.76770862255072));
#76024=CARTESIAN_POINT('Ctrl Pts',(-17.4914348451035,-17.2380097651368,
-4.76690910674101));
#76025=CARTESIAN_POINT('Ctrl Pts',(-17.4966682387519,-17.2342279535976,
-4.76652349030325));
#76026=CARTESIAN_POINT('Ctrl Pts',(-17.508794111383,-17.2255495922055,-4.76563507308644));
#76027=CARTESIAN_POINT('Ctrl Pts',(-17.5156988144551,-17.2206702496235,
-4.76513293835758));
#76028=CARTESIAN_POINT('Ctrl Pts',(-17.5343516609808,-17.207655694599,-4.76378634062934));
#76029=CARTESIAN_POINT('Ctrl Pts',(-17.5461533760406,-17.1995977613702,
-4.76294481895271));
#76030=CARTESIAN_POINT('Ctrl Pts',(-17.6551776126149,-17.1267660568906,
-4.7552637544997));
#76031=CARTESIAN_POINT('Ctrl Pts',(-17.7575297815945,-17.0700202272178,
-4.7487408193637));
#76032=CARTESIAN_POINT('Ctrl Pts',(-18.0124223312777,-16.9551273613875,
-4.73343473580252));
#76033=CARTESIAN_POINT('Ctrl Pts',(-18.1679887777992,-16.9055899459226,
-4.72483467487124));
#76034=CARTESIAN_POINT('Ctrl Pts',(-18.3595755969936,-16.8681208820909,
-4.713625662658));
#76035=CARTESIAN_POINT('Ctrl Pts',(-18.3916173547746,-16.8626173939183,
-4.7117296076978));
#76036=CARTESIAN_POINT('Ctrl Pts',(-18.4309325495454,-16.8567932004747,
-4.70936319797136));
#76037=CARTESIAN_POINT('Ctrl Pts',(-18.4380993054476,-16.855769051888,-4.70893020995935));
#76038=CARTESIAN_POINT('Ctrl Pts',(-18.4493423561248,-16.8542211948253,
-4.70824821888843));
#76039=CARTESIAN_POINT('Ctrl Pts',(-18.4534152406589,-16.8536725513348,
-4.70800060161163));
#76040=CARTESIAN_POINT('Ctrl Pts',(-18.4610310011228,-16.8526692293886,
-4.70753649923065));
#76041=CARTESIAN_POINT('Ctrl Pts',(-18.4645734390048,-16.8522116567716,
-4.70732017949619));
#76042=CARTESIAN_POINT('Ctrl Pts',(-18.4726622399494,-16.8511876415534,
-4.70682522962215));
#76043=CARTESIAN_POINT('Ctrl Pts',(-18.4772092785096,-16.8506269929698,
-4.70654627760946));
#76044=CARTESIAN_POINT('Ctrl Pts',(-18.4911906232533,-16.8489491538935,
-4.70568640953065));
#76045=CARTESIAN_POINT('Ctrl Pts',(-18.5006305072274,-16.8478807241849,
-4.70510285426571));
#76046=CARTESIAN_POINT('Ctrl Pts',(-18.5854821663644,-16.8388550173133,
-4.69983257637252));
#76047=CARTESIAN_POINT('Ctrl Pts',(-18.6612558909031,-16.8348922985301,
-4.69495116258859));
#76048=CARTESIAN_POINT('Ctrl Pts',(-18.9219988317722,-16.835270365541,-4.67789831655831));
#76049=CARTESIAN_POINT('Ctrl Pts',(-19.1061355323877,-16.8597708283004,
-4.66550103539425));
#76050=CARTESIAN_POINT('Ctrl Pts',(-19.3361766263971,-16.9217514690625,
-4.65047362438357));
#76051=CARTESIAN_POINT('Ctrl Pts',(-19.387066148928,-16.9375444431611,-4.64717204461378));
#76052=CARTESIAN_POINT('Ctrl Pts',(-19.4491379036165,-16.9594077070313,
-4.64317037238864));
#76053=CARTESIAN_POINT('Ctrl Pts',(-19.460929182786,-16.9636790397394,-4.64241132003099));
#76054=CARTESIAN_POINT('Ctrl Pts',(-19.4795054404177,-16.9705955355016,
-4.64121709005571));
#76055=CARTESIAN_POINT('Ctrl Pts',(-19.4863157803131,-16.9731713105016,
-4.64077960867383));
#76056=CARTESIAN_POINT('Ctrl Pts',(-19.4990579101942,-16.9780658688821,
-4.63996167685359));
#76057=CARTESIAN_POINT('Ctrl Pts',(-19.5049927715524,-16.9803763778228,
-4.63958095452098));
#76058=CARTESIAN_POINT('Ctrl Pts',(-19.5182499976492,-16.9856065804052,
-4.63873100461963));
#76059=CARTESIAN_POINT('Ctrl Pts',(-19.5255666877404,-16.9885404712933,
-4.63826226086022));
#76060=CARTESIAN_POINT('Ctrl Pts',(-19.5440619743999,-16.9960770113323,
-4.63707813758241));
#76061=CARTESIAN_POINT('Ctrl Pts',(-19.5552179418437,-17.0007347076697,
-4.63636462361637));
#76062=CARTESIAN_POINT('Ctrl Pts',(-19.6186385932735,-17.0278535395828,
-4.63231158884045));
#76063=CARTESIAN_POINT('Ctrl Pts',(-19.6700237506961,-17.0523196556421,
-4.62904117540495));
#76064=CARTESIAN_POINT('Ctrl Pts',(-19.7441234589785,-17.0913386639317,
-4.62431037108652));
#76065=CARTESIAN_POINT('Ctrl Pts',(-19.767642783662,-17.1043007076207,-4.62280637074052));
#76066=CARTESIAN_POINT('Ctrl Pts',(-19.891285029825,-17.1755427024923,-4.61486888328844));
#76067=CARTESIAN_POINT('Ctrl Pts',(-19.9867433515099,-17.2415193516592,
-4.60864395678167));
#76068=CARTESIAN_POINT('Ctrl Pts',(-20.1382163806034,-17.3657241310027,
-4.5979650732624));
#76069=CARTESIAN_POINT('Ctrl Pts',(-20.1971739750625,-17.4199377643235,
-4.59356330534814));
#76070=CARTESIAN_POINT('Ctrl Pts',(-20.277994046911,-17.5031841055979,-4.58692635700263));
#76071=CARTESIAN_POINT('Ctrl Pts',(-20.3024071368253,-17.5296484899652,
-4.58483223435928));
#76072=CARTESIAN_POINT('Ctrl Pts',(-20.3310517233175,-17.5623343884094,
-4.58224580120193));
#76073=CARTESIAN_POINT('Ctrl Pts',(-20.3359416520772,-17.5679741120326,
-4.58179952928709));
#76074=CARTESIAN_POINT('Ctrl Pts',(-20.3435094238394,-17.5767961200587,
-4.58110122599477));
#76075=CARTESIAN_POINT('Ctrl Pts',(-20.3462079433198,-17.5799606989424,
-4.58085069169639));
#76076=CARTESIAN_POINT('Ctrl Pts',(-20.3512028583503,-17.5858533640531,
-4.58038405528615));
#76077=CARTESIAN_POINT('Ctrl Pts',(-20.3535016924873,-17.5885793079941,
-4.58016813662203));
#76078=CARTESIAN_POINT('Ctrl Pts',(-20.3586930848236,-17.5947668845043,
-4.57967791240857));
#76079=CARTESIAN_POINT('Ctrl Pts',(-20.3615814577661,-17.598231944853,-4.57940330915237));
#76080=CARTESIAN_POINT('Ctrl Pts',(-20.3701034741884,-17.6085221465587,
-4.5785876626009));
#76081=CARTESIAN_POINT('Ctrl Pts',(-20.3757053375998,-17.6153733134639,
-4.57804440659786));
#76082=CARTESIAN_POINT('Ctrl Pts',(-20.4168972455648,-17.666401264886,-4.57399800027048));
#76083=CARTESIAN_POINT('Ctrl Pts',(-20.4507385734215,-17.7119537513666,
-4.57038515258016));
#76084=CARTESIAN_POINT('Ctrl Pts',(-20.5175961194107,-17.8099379597198,
-4.56270245993221));
#76085=CARTESIAN_POINT('Ctrl Pts',(-20.5502246796521,-17.862574398703,-4.55862482500236));
#76086=CARTESIAN_POINT('Ctrl Pts',(-20.6341054045249,-18.0121591340198,
-4.54729669943314));
#76087=CARTESIAN_POINT('Ctrl Pts',(-20.6802113236659,-18.1117819658407,
-4.54004811994042));
#76088=CARTESIAN_POINT('Ctrl Pts',(-20.737683337339,-18.2664292201099,-4.52944129938011));
#76089=CARTESIAN_POINT('Ctrl Pts',(-20.7549277316741,-18.3190654488591,
-4.52593479478235));
#76090=CARTESIAN_POINT('Ctrl Pts',(-20.7795153219938,-18.4054279742752,
-4.52035281203362));
#76091=CARTESIAN_POINT('Ctrl Pts',(-20.7881324592452,-18.4387612930963,
-4.51823847279913));
#76092=CARTESIAN_POINT('Ctrl Pts',(-20.7983855428401,-18.4828321739193,
-4.5154938061602));
#76093=CARTESIAN_POINT('Ctrl Pts',(-20.8007569915616,-18.493391601517,-4.51483996346439));
#76094=CARTESIAN_POINT('Ctrl Pts',(-20.8045078950316,-18.5107136069883,
-4.5137734466202));
#76095=CARTESIAN_POINT('Ctrl Pts',(-20.8059354161052,-18.5174654705448,
-4.51335923738922));
#76096=CARTESIAN_POINT('Ctrl Pts',(-20.8086343584915,-18.5305466189247,
-4.51255960765106));
#76097=CARTESIAN_POINT('Ctrl Pts',(-20.8099098928332,-18.5368749680933,
-4.51217405953265));
#76098=CARTESIAN_POINT('Ctrl Pts',(-20.8127876276471,-18.5514973718676,
-4.51128614295279));
#76099=CARTESIAN_POINT('Ctrl Pts',(-20.8143691793942,-18.5597954148903,
-4.51078443813165));
#76100=CARTESIAN_POINT('Ctrl Pts',(-20.8184877291796,-18.5821305946227,
-4.50943975416288));
#76101=CARTESIAN_POINT('Ctrl Pts',(-20.8209326205792,-18.5961844268039,
-4.50859970311708));
#76102=CARTESIAN_POINT('Ctrl Pts',(-20.8418093118175,-18.7238153633244,
-4.50102303982116));
#76103=CARTESIAN_POINT('Ctrl Pts',(-20.8510962905331,-18.83870077858,-4.49459283785146));
#76104=CARTESIAN_POINT('Ctrl Pts',(-20.8508421940249,-19.1400360575658,
-4.47808641480517));
#76105=CARTESIAN_POINT('Ctrl Pts',(-20.8261075481251,-19.3254189869919,
-4.46831883007838));
#76106=CARTESIAN_POINT('Ctrl Pts',(-20.7737437540471,-19.5188655758418,
-4.45654187285768));
#76107=CARTESIAN_POINT('Ctrl Pts',(-20.7698906309532,-19.5325518732858,
-4.45569948325786));
#76108=CARTESIAN_POINT('Ctrl Pts',(-20.7643392700573,-19.5515351286692,
-4.45451694403742));
#76109=CARTESIAN_POINT('Ctrl Pts',(-20.7627574775556,-19.5568661155281,
-4.45418329897582));
#76110=CARTESIAN_POINT('Ctrl Pts',(-20.7601843572481,-19.5654144474497,
-4.45364569800847));
#76111=CARTESIAN_POINT('Ctrl Pts',(-20.7592063133213,-19.5686358098699,
-4.45344251465341));
#76112=CARTESIAN_POINT('Ctrl Pts',(-20.7571469227646,-19.5753610313025,
-4.45301706305863));
#76113=CARTESIAN_POINT('Ctrl Pts',(-20.7560641558258,-19.5788644155073,
-4.45279470933072));
#76114=CARTESIAN_POINT('Ctrl Pts',(-20.7534222730193,-19.5873343854775,
-4.45225541434439));
#76115=CARTESIAN_POINT('Ctrl Pts',(-20.7518539349012,-19.5922980510786,
-4.4519379369362));
#76116=CARTESIAN_POINT('Ctrl Pts',(-20.7463005708686,-19.6096509614781,
-4.45082314131569));
#76117=CARTESIAN_POINT('Ctrl Pts',(-20.7422197134157,-19.622008908838,-4.4500204769994));
#76118=CARTESIAN_POINT('Ctrl Pts',(-20.7330366644334,-19.6489798965801,
-4.44825065621382));
#76119=CARTESIAN_POINT('Ctrl Pts',(-20.7278880804562,-19.6635748542383,
-4.44728126432251));
#76120=CARTESIAN_POINT('Ctrl Pts',(-20.7225805839746,-19.678110364228,-4.44630500845845));
#76121=CARTESIAN_POINT('Origin',(-18.734,-18.952,0.));
#76122=CARTESIAN_POINT('',(-20.7225805821191,-19.6781103693095,-3.64442446878243));
#76123=CARTESIAN_POINT('',(-20.7225805144725,-19.6781105545716,-3.86819367631211));
#76124=CARTESIAN_POINT('',(-20.7225805821191,-19.6781103693095,0.));
#76125=CARTESIAN_POINT('',(-20.850999091379,-18.950054148737,-3.9109852266757));
#76126=CARTESIAN_POINT('Ctrl Pts',(-20.7225805144725,-19.6781105545716,
-3.86819367631211));
#76127=CARTESIAN_POINT('Ctrl Pts',(-20.7339917000002,-19.6468590308957,
-3.87027308349242));
#76128=CARTESIAN_POINT('Ctrl Pts',(-20.7446699030894,-19.6153283311154,
-3.87233005795932));
#76129=CARTESIAN_POINT('Ctrl Pts',(-20.759305937768,-19.5685008207448,-3.87532605152801));
#76130=CARTESIAN_POINT('Ctrl Pts',(-20.7638396682874,-19.5534053089804,
-3.87628298861571));
#76131=CARTESIAN_POINT('Ctrl Pts',(-20.7704398408054,-19.5305040451152,
-3.87772167942554));
#76132=CARTESIAN_POINT('Ctrl Pts',(-20.7726308327077,-19.5227350402634,
-3.87820748126762));
#76133=CARTESIAN_POINT('Ctrl Pts',(-20.7764754410657,-19.508797853311,-3.87907500430636));
#76134=CARTESIAN_POINT('Ctrl Pts',(-20.7781456752986,-19.5026343944495,
-3.87945726175366));
#76135=CARTESIAN_POINT('Ctrl Pts',(-20.7816285950472,-19.4895475364464,
-3.88026600625009));
#76136=CARTESIAN_POINT('Ctrl Pts',(-20.7834341154902,-19.4826223001252,
-3.88069225692262));
#76137=CARTESIAN_POINT('Ctrl Pts',(-20.7870374715709,-19.4685085137492,
-3.88155753403966));
#76138=CARTESIAN_POINT('Ctrl Pts',(-20.7888327535059,-19.461319410277,-3.88199647325397));
#76139=CARTESIAN_POINT('Ctrl Pts',(-20.7932121438162,-19.4433822751305,
-3.88308724193768));
#76140=CARTESIAN_POINT('Ctrl Pts',(-20.7957499029133,-19.4326230729711,
-3.88373758668791));
#76141=CARTESIAN_POINT('Ctrl Pts',(-20.8334343576381,-19.2670610545227,
-3.89368680767375));
#76142=CARTESIAN_POINT('Ctrl Pts',(-20.8511450351567,-19.1088094550095,
-3.90236296950705));
#76143=CARTESIAN_POINT('Ctrl Pts',(-20.8509991056246,-18.9500540337685,
-3.91098525629469));
#76144=CARTESIAN_POINT('Ctrl Pts',(-20.8509991057315,-18.9500541499897,
-3.91098524998252));
#76145=CARTESIAN_POINT('Ctrl Pts',(-20.8508677552328,-18.8071505928033,
-3.91874659410215));
#76146=CARTESIAN_POINT('Ctrl Pts',(-20.8362671717988,-18.6646421546169,
-3.9264424364072));
#76147=CARTESIAN_POINT('Ctrl Pts',(-20.8054602107921,-18.5151512492231,
-3.93541352843948));
#76148=CARTESIAN_POINT('Ctrl Pts',(-20.8034244703783,-18.5056071353841,
-3.93599034923015));
#76149=CARTESIAN_POINT('Ctrl Pts',(-20.8001174997672,-18.4906120914082,
-3.93690350748031));
#76150=CARTESIAN_POINT('Ctrl Pts',(-20.7988904876265,-18.4851514189999,
-3.93723749209016));
#76151=CARTESIAN_POINT('Ctrl Pts',(-20.7965251623796,-18.4748165890272,
-3.93787243749969));
#76152=CARTESIAN_POINT('Ctrl Pts',(-20.795391185985,-18.4699414658693,-3.93817315633918));
#76153=CARTESIAN_POINT('Ctrl Pts',(-20.7934048895302,-18.4615372779484,
-3.93869371378611));
#76154=CARTESIAN_POINT('Ctrl Pts',(-20.7925607518292,-18.458006263577,-3.93891308271453));
#76155=CARTESIAN_POINT('Ctrl Pts',(-20.7909045653938,-18.4511564288955,
-3.93933994041501));
#76156=CARTESIAN_POINT('Ctrl Pts',(-20.7900935637945,-18.4478373968713,
-3.93954736266223));
#76157=CARTESIAN_POINT('Ctrl Pts',(-20.7878796792858,-18.4388712429774,
-3.94010927374737));
#76158=CARTESIAN_POINT('Ctrl Pts',(-20.7864615548879,-18.4332279670829,
-3.94046462818654));
#76159=CARTESIAN_POINT('Ctrl Pts',(-20.7810870799278,-18.4122078279738,
-3.94179437413913));
#76160=CARTESIAN_POINT('Ctrl Pts',(-20.7769811546349,-18.396870223128,-3.9427768674802));
#76161=CARTESIAN_POINT('Ctrl Pts',(-20.7391408561341,-18.2616273392847,
-3.95153986855596));
#76162=CARTESIAN_POINT('Ctrl Pts',(-20.6950603853006,-18.1448812701311,
-3.95978535644781));
#76163=CARTESIAN_POINT('Ctrl Pts',(-20.6100511858113,-17.96853979006,-3.97272142857487));
#76164=CARTESIAN_POINT('Ctrl Pts',(-20.5759023984443,-17.905979727209,-3.97741812474979));
#76165=CARTESIAN_POINT('Ctrl Pts',(-20.4894057397083,-17.7649374867526,
-3.98816741794171));
#76166=CARTESIAN_POINT('Ctrl Pts',(-20.4348357081262,-17.6879870599765,
-3.99415326834526));
#76167=CARTESIAN_POINT('Ctrl Pts',(-20.3617156831655,-17.5982296750814,
-4.00126722239978));
#76168=CARTESIAN_POINT('Ctrl Pts',(-20.3478648540158,-17.5817472041432,
-4.0025798484107));
#76169=CARTESIAN_POINT('Ctrl Pts',(-20.3291372683196,-17.5601393702983,
-4.00430963397666));
#76170=CARTESIAN_POINT('Ctrl Pts',(-20.3244831877986,-17.5548235084573,
-4.00473592830462));
#76171=CARTESIAN_POINT('Ctrl Pts',(-20.3152194689624,-17.5443488179071,
-4.00557743634176));
#76172=CARTESIAN_POINT('Ctrl Pts',(-20.3106109842,-17.5391890905926,-4.00599269058446));
#76173=CARTESIAN_POINT('Ctrl Pts',(-20.3016578333715,-17.5292633744369,
-4.00679298141101));
#76174=CARTESIAN_POINT('Ctrl Pts',(-20.2973165252565,-17.5244944723293,
-4.00717815273047));
#76175=CARTESIAN_POINT('Ctrl Pts',(-20.2872662273235,-17.5135551134005,
-4.00806327701928));
#76176=CARTESIAN_POINT('Ctrl Pts',(-20.2815421165878,-17.5073986483377,
-4.00856257979323));
#76177=CARTESIAN_POINT('Ctrl Pts',(-20.2661032197986,-17.4909906958999,
-4.009896588182));
#76178=CARTESIAN_POINT('Ctrl Pts',(-20.2563221612917,-17.4808019458866,
-4.01072843890351));
#76179=CARTESIAN_POINT('Ctrl Pts',(-20.1714442557834,-17.3941390664928,
-4.01783640143235));
#76180=CARTESIAN_POINT('Ctrl Pts',(-20.0907374091159,-17.3233672534982,
-4.02384940625994));
#76181=CARTESIAN_POINT('Ctrl Pts',(-19.9105739166692,-17.1881103556605,
-4.03622626818153));
#76182=CARTESIAN_POINT('Ctrl Pts',(-19.8103776060796,-17.1252425182423,
-4.04254151760226));
#76183=CARTESIAN_POINT('Ctrl Pts',(-19.6539374711222,-17.0444446560424,
-4.05224819475398));
#76184=CARTESIAN_POINT('Ctrl Pts',(-19.6013415514799,-17.0199622104733,
-4.05549044429343));
#76185=CARTESIAN_POINT('Ctrl Pts',(-19.5207342985949,-16.9863961669037,
-4.06052168939224));
#76186=CARTESIAN_POINT('Ctrl Pts',(-19.493427583706,-16.9756855424803,-4.06223656050007));
#76187=CARTESIAN_POINT('Ctrl Pts',(-19.4593546534484,-16.9631313731406,
-4.0643995491408));
#76188=CARTESIAN_POINT('Ctrl Pts',(-19.4527887179666,-16.9607489952267,
-4.0648174171707));
#76189=CARTESIAN_POINT('Ctrl Pts',(-19.4423642044375,-16.9570248517356,
-4.06548270052494));
#76190=CARTESIAN_POINT('Ctrl Pts',(-19.4385132587242,-16.9556616629554,
-4.06572886278131));
#76191=CARTESIAN_POINT('Ctrl Pts',(-19.4312842020671,-16.9531261851919,
-4.06619175108062));
#76192=CARTESIAN_POINT('Ctrl Pts',(-19.4279070585022,-16.951951305728,-4.06640832093716));
#76193=CARTESIAN_POINT('Ctrl Pts',(-19.4201600771924,-16.9492781799044,
-4.06690585590914));
#76194=CARTESIAN_POINT('Ctrl Pts',(-19.4157883136037,-16.9477856814404,
-4.06718715590882));
#76195=CARTESIAN_POINT('Ctrl Pts',(-19.4022263801768,-16.9432052120397,
-4.06806136367723));
#76196=CARTESIAN_POINT('Ctrl Pts',(-19.3930200083535,-16.9401661063384,
-4.06865703730769));
#76197=CARTESIAN_POINT('Ctrl Pts',(-19.2895324269085,-16.9067904780016,
-4.07537527310461));
#76198=CARTESIAN_POINT('Ctrl Pts',(-19.193265016635,-16.8830463379857,-4.08182716728371));
#76199=CARTESIAN_POINT('Ctrl Pts',(-18.929784823183,-16.8373572780874,-4.09944296715288));
#76200=CARTESIAN_POINT('Ctrl Pts',(-18.7609960367477,-16.8284808495551,
-4.11062975816369));
#76201=CARTESIAN_POINT('Ctrl Pts',(-18.5459926054869,-16.8428402538046,
-4.12416079473513));
#76202=CARTESIAN_POINT('Ctrl Pts',(-18.4991735865144,-16.8475383767336,
-4.12706847298146));
#76203=CARTESIAN_POINT('Ctrl Pts',(-18.4408421272215,-16.855362947944,-4.13064512008699));
#76204=CARTESIAN_POINT('Ctrl Pts',(-18.4291505339283,-16.8570309600565,
-4.13135970110613));
#76205=CARTESIAN_POINT('Ctrl Pts',(-18.4102896003126,-16.8598830426988,
-4.13250889118889));
#76206=CARTESIAN_POINT('Ctrl Pts',(-18.4031114500929,-16.8610063234234,
-4.13294541500388));
#76207=CARTESIAN_POINT('Ctrl Pts',(-18.3896505484418,-16.863183819332,-4.13376248271698));
#76208=CARTESIAN_POINT('Ctrl Pts',(-18.3833665138931,-16.8642294807137,
-4.13414329298243));
#76209=CARTESIAN_POINT('Ctrl Pts',(-18.3692954875216,-16.8666362173132,
-4.13499462928351));
#76210=CARTESIAN_POINT('Ctrl Pts',(-18.3615111799843,-16.8680125794238,
-4.13546466425508));
#76211=CARTESIAN_POINT('Ctrl Pts',(-18.3417722729069,-16.8716167948235,
-4.13665426541073));
#76212=CARTESIAN_POINT('Ctrl Pts',(-18.3298287233502,-16.873904126691,-4.13737193548605));
#76213=CARTESIAN_POINT('Ctrl Pts',(-18.2610582986873,-16.8876898021478,
-4.1414928921393));
#76214=CARTESIAN_POINT('Ctrl Pts',(-18.2047002031986,-16.901416413084,-4.14482426033528));
#76215=CARTESIAN_POINT('Ctrl Pts',(-17.9819385892691,-16.9654703850837,
-4.15790804927205));
#76216=CARTESIAN_POINT('Ctrl Pts',(-17.8214651537316,-17.0338826082114,
-4.16708455584795));
#76217=CARTESIAN_POINT('Ctrl Pts',(-17.6227131093607,-17.149260852885,-4.179771905794));
#76218=CARTESIAN_POINT('Ctrl Pts',(-17.5754054539349,-17.1792945009904,
-4.18290877768369));
#76219=CARTESIAN_POINT('Ctrl Pts',(-17.5057219806043,-17.2275152709477,
-4.18779537036499));
#76220=CARTESIAN_POINT('Ctrl Pts',(-17.4824326783955,-17.2443426781843,
-4.18947613929834));
#76221=CARTESIAN_POINT('Ctrl Pts',(-17.4539345386543,-17.2658298131928,
-4.19160254512058));
#76222=CARTESIAN_POINT('Ctrl Pts',(-17.4483955439157,-17.2700491494604,
-4.19201918815838));
#76223=CARTESIAN_POINT('Ctrl Pts',(-17.4396690466386,-17.2767648599085,
-4.19268108617326));
#76224=CARTESIAN_POINT('Ctrl Pts',(-17.4364676607751,-17.2792432276448,
-4.19292508720424));
#76225=CARTESIAN_POINT('Ctrl Pts',(-17.4304468926759,-17.2839319165853,
-4.19338624156579));
#76226=CARTESIAN_POINT('Ctrl Pts',(-17.4276260047776,-17.2861402164602,
-4.19360325259075));
#76227=CARTESIAN_POINT('Ctrl Pts',(-17.421194077331,-17.291201761179,-4.19410021849645));
#76228=CARTESIAN_POINT('Ctrl Pts',(-17.4175867325698,-17.2940596243904,
-4.19438050036752));
#76229=CARTESIAN_POINT('Ctrl Pts',(-17.4080439837439,-17.301670498524,-4.19512602741155));
#76230=CARTESIAN_POINT('Ctrl Pts',(-17.4021248829129,-17.3064437144276,
-4.19559266622832));
#76231=CARTESIAN_POINT('Ctrl Pts',(-17.3611207346591,-17.3398759879602,
-4.19885391415649));
#76232=CARTESIAN_POINT('Ctrl Pts',(-17.3269404522327,-17.3696207571177,
-4.20171901078609));
#76233=CARTESIAN_POINT('Ctrl Pts',(-17.2894212158693,-17.4044484127776,
-4.20500893655988));
#76234=CARTESIAN_POINT('Ctrl Pts',(-17.2851158301567,-17.4084785586425,
-4.2053887019268));
#76235=CARTESIAN_POINT('Ctrl Pts',(-17.2636231234322,-17.4287664137077,
-4.20729555781074));
#76236=CARTESIAN_POINT('Ctrl Pts',(-17.2466927464502,-17.4452930634201,
-4.20883323813897));
#76237=CARTESIAN_POINT('Ctrl Pts',(-17.1284398755276,-17.5646615671128,
-4.21981020068044));
#76238=CARTESIAN_POINT('Ctrl Pts',(-17.0375844448488,-17.6773586527658,
-4.22947212622353));
#76239=CARTESIAN_POINT('Ctrl Pts',(-16.9252306107284,-17.8502460464882,
-4.24279355778659));
#76240=CARTESIAN_POINT('Ctrl Pts',(-16.8938372374362,-17.9035198546591,
-4.2467246209479));
#76241=CARTESIAN_POINT('Ctrl Pts',(-16.8473267330603,-17.9909896167273,
-4.25289751514259));
#76242=CARTESIAN_POINT('Ctrl Pts',(-16.8307063098121,-18.0243414537257,
-4.25518924739902));
#76243=CARTESIAN_POINT('Ctrl Pts',(-16.8102724707932,-18.0682096558271,
-4.25812611102926));
#76244=CARTESIAN_POINT('Ctrl Pts',(-16.8056506283698,-18.0783400619033,
-4.25879906924924));
#76245=CARTESIAN_POINT('Ctrl Pts',(-16.7982659483824,-18.0948703362515,
-4.25988879295217));
#76246=CARTESIAN_POINT('Ctrl Pts',(-16.7954544592642,-18.1012481164458,
-4.26030722416042));
#76247=CARTESIAN_POINT('Ctrl Pts',(-16.7901095978453,-18.1135368468801,
-4.26110964456268));
#76248=CARTESIAN_POINT('Ctrl Pts',(-16.7875715653679,-18.1194456744491,
-4.26149378964269));
#76249=CARTESIAN_POINT('Ctrl Pts',(-16.781823763534,-18.1329971597848,-4.26237099455689));
#76250=CARTESIAN_POINT('Ctrl Pts',(-16.7786318656496,-18.1406473191925,
-4.26286344239535));
#76251=CARTESIAN_POINT('Ctrl Pts',(-16.7702752310087,-18.1610117871001,
-4.2641671427367));
#76252=CARTESIAN_POINT('Ctrl Pts',(-16.7651889943345,-18.1737580334519,
-4.26497574320061));
#76253=CARTESIAN_POINT('Ctrl Pts',(-16.7275795357931,-18.2707373687653,
-4.27107396391681));
#76254=CARTESIAN_POINT('Ctrl Pts',(-16.700349111353,-18.3569295994903,-4.27618099605698));
#76255=CARTESIAN_POINT('Ctrl Pts',(-16.6452676424002,-18.5800477179326,
-4.28890311167347));
#76256=CARTESIAN_POINT('Ctrl Pts',(-16.6253021079877,-18.7184562078926,
-4.29632347502236));
#76257=CARTESIAN_POINT('Ctrl Pts',(-16.6166375322596,-18.9130256558026,
-4.30708178341982));
#76258=CARTESIAN_POINT('Ctrl Pts',(-16.6163418218673,-18.968303707417,-4.31017826428166));
#76259=CARTESIAN_POINT('Ctrl Pts',(-16.6191706651434,-19.0519831320674,
-4.31500785401755));
#76260=CARTESIAN_POINT('Ctrl Pts',(-16.6207066568436,-19.08041654205,-4.31667390547102));
#76261=CARTESIAN_POINT('Ctrl Pts',(-16.6233297507466,-19.1157324064544,
-4.31878386147019));
#76262=CARTESIAN_POINT('Ctrl Pts',(-16.6238780581976,-19.1226534197843,
-4.31919930486241));
#76263=CARTESIAN_POINT('Ctrl Pts',(-16.6247996081737,-19.1336013825182,
-4.31985972740497));
#76264=CARTESIAN_POINT('Ctrl Pts',(-16.6251503689035,-19.1376302448607,
-4.32010346206463));
#76265=CARTESIAN_POINT('Ctrl Pts',(-16.6258337042167,-19.1452270958155,
-4.32056440891715));
#76266=CARTESIAN_POINT('Ctrl Pts',(-16.6261637946523,-19.1487952538634,
-4.32078148053715));
#76267=CARTESIAN_POINT('Ctrl Pts',(-16.6269392326948,-19.1569516359477,
-4.3212789704458));
#76268=CARTESIAN_POINT('Ctrl Pts',(-16.6273905078855,-19.1615392493075,
-4.32155971824884));
#76269=CARTESIAN_POINT('Ctrl Pts',(-16.6286284567157,-19.1737157531584,
-4.32230728971806));
#76270=CARTESIAN_POINT('Ctrl Pts',(-16.6294411698588,-19.1813018467447,
-4.32277551896893));
#76271=CARTESIAN_POINT('Ctrl Pts',(-16.6354230540826,-19.2344255718266,
-4.32607105529165));
#76272=CARTESIAN_POINT('Ctrl Pts',(-16.6420283922313,-19.2797857598849,
-4.32897049370731));
#76273=CARTESIAN_POINT('Ctrl Pts',(-16.6567510987132,-19.3620633594794,
-4.33434424974106));
#76274=CARTESIAN_POINT('Ctrl Pts',(-16.6643956519628,-19.3990487341738,
-4.33680275869016));
#76275=CARTESIAN_POINT('Ctrl Pts',(-16.703903744442,-19.5673492742669,-4.34813514041002));
#76276=CARTESIAN_POINT('Ctrl Pts',(-16.747308258994,-19.6956436502566,-4.35715618972546));
#76277=CARTESIAN_POINT('Ctrl Pts',(-16.8280764553227,-19.8755804272229,
-4.36990178836925));
#76278=CARTESIAN_POINT('Ctrl Pts',(-16.8559888461057,-19.9310917295683,
-4.3738525506462));
#76279=CARTESIAN_POINT('Ctrl Pts',(-16.9045504775818,-20.0179272672908,
-4.38005259591364));
#76280=CARTESIAN_POINT('Ctrl Pts',(-16.9236588781968,-20.0500673004922,
-4.3823523257157));
#76281=CARTESIAN_POINT('Ctrl Pts',(-16.9495583751451,-20.0911142910218,
-4.38529781204679));
#76282=CARTESIAN_POINT('Ctrl Pts',(-16.9555817670222,-20.10049548392,-4.38597159802395));
#76283=CARTESIAN_POINT('Ctrl Pts',(-16.9654926666097,-20.1156663750822,
-4.38706232698372));
#76284=CARTESIAN_POINT('Ctrl Pts',(-16.9693351123407,-20.1214851246701,
-4.3874809414376));
#76285=CARTESIAN_POINT('Ctrl Pts',(-16.9767758776042,-20.1326327651176,
-4.38828348979272));
#76286=CARTESIAN_POINT('Ctrl Pts',(-16.9803698579053,-20.1379644465768,
-4.38866758077857));
#76287=CARTESIAN_POINT('Ctrl Pts',(-16.9886489814745,-20.1501266319347,
-4.38954435320516));
#76288=CARTESIAN_POINT('Ctrl Pts',(-16.9933500509916,-20.1569462071033,
-4.39003642474036));
#76289=CARTESIAN_POINT('Ctrl Pts',(-17.0059334137057,-20.174972851478,-4.39133846794334));
#76290=CARTESIAN_POINT('Ctrl Pts',(-17.0138847678329,-20.1861314044111,
-4.39214579845206));
#76291=CARTESIAN_POINT('Ctrl Pts',(-17.0745473175795,-20.2695370136281,
-4.39819239748218));
#76292=CARTESIAN_POINT('Ctrl Pts',(-17.131684041257,-20.3384607291917,-4.40325275680924));
#76293=CARTESIAN_POINT('Ctrl Pts',(-17.288727770133,-20.5051780945823,-4.41593712263578));
#76294=CARTESIAN_POINT('Ctrl Pts',(-17.3942502941685,-20.5970662521818,
-4.42336238006537));
#76295=CARTESIAN_POINT('Ctrl Pts',(-17.5535787635507,-20.7102417494571,
-4.43415301056376));
#76296=CARTESIAN_POINT('Ctrl Pts',(-17.6003707804107,-20.7407683657582,
-4.43728098721985));
#76297=CARTESIAN_POINT('Ctrl Pts',(-17.6729278130065,-20.784112725906,-4.44215503288807));
#76298=CARTESIAN_POINT('Ctrl Pts',(-17.6978392325704,-20.798315765815,-4.44383256947258));
#76299=CARTESIAN_POINT('Ctrl Pts',(-17.7291438673546,-20.8153307744653,
-4.44595536300871));
#76300=CARTESIAN_POINT('Ctrl Pts',(-17.735273998735,-20.8186236347251,-4.44637174353714));
#76301=CARTESIAN_POINT('Ctrl Pts',(-17.7449953287191,-20.8237839468382,
-4.44703331869259));
#76302=CARTESIAN_POINT('Ctrl Pts',(-17.7485759027929,-20.8256714577183,
-4.4472772614451));
#76303=CARTESIAN_POINT('Ctrl Pts',(-17.7553359429512,-20.8292102970675,
-4.44773837028484));
#76304=CARTESIAN_POINT('Ctrl Pts',(-17.758514195629,-20.8308638270862,-4.44795539444513));
#76305=CARTESIAN_POINT('Ctrl Pts',(-17.7657862001301,-20.8346237631418,
-4.44845247445339));
#76306=CARTESIAN_POINT('Ctrl Pts',(-17.7698826306683,-20.8367248852377,
-4.44873285784151));
#76307=CARTESIAN_POINT('Ctrl Pts',(-17.7807679828604,-20.8422633749844,
-4.44947883016849));
#76308=CARTESIAN_POINT('Ctrl Pts',(-17.7875685683302,-20.8456774927272,
-4.44994581534779));
#76309=CARTESIAN_POINT('Ctrl Pts',(-17.8350857344075,-20.869212781581,-4.45321451189403));
#76310=CARTESIAN_POINT('Ctrl Pts',(-17.8764191311835,-20.8880542573626,
-4.45608706631556));
#76311=CARTESIAN_POINT('Ctrl Pts',(-17.9236576980185,-20.9077780490075,
-4.45937718209051));
#76312=CARTESIAN_POINT('Ctrl Pts',(-17.9290016899543,-20.9099836932757,
-4.45974949026986));
#76313=CARTESIAN_POINT('Ctrl Pts',(-18.0801810755522,-20.971656945802,-4.47028367104066));
#76314=CARTESIAN_POINT('Ctrl Pts',(-18.232190867034,-21.014688697066,-4.48087398619109));
#76315=CARTESIAN_POINT('Ctrl Pts',(-18.4891812364084,-21.057317310925,-4.49778554889153));
#76316=CARTESIAN_POINT('Ctrl Pts',(-18.5918946355419,-21.0667360916899,
-4.50430475197365));
#76317=CARTESIAN_POINT('Ctrl Pts',(-18.7097046862916,-21.0689123739475,
-4.51149034843639));
#76318=CARTESIAN_POINT('Ctrl Pts',(-18.7245123799087,-21.0690305297247,
-4.51238847350152));
#76319=CARTESIAN_POINT('Ctrl Pts',(-18.7470890259737,-21.0689737904363,
-4.51375036900016));
#76320=CARTESIAN_POINT('Ctrl Pts',(-18.7548575690699,-21.0689115041298,
-4.51421765079908));
#76321=CARTESIAN_POINT('Ctrl Pts',(-18.76898648262,-21.0687204381559,-4.51506512559451));
#76322=CARTESIAN_POINT('Ctrl Pts',(-18.7753469232033,-21.0686057499172,
-4.51544575524532));
#76323=CARTESIAN_POINT('Ctrl Pts',(-18.789072577685,-21.0682963623672,-4.51626528409207));
#76324=CARTESIAN_POINT('Ctrl Pts',(-18.7964375041551,-21.0680918794704,
-4.51670387194656));
#76325=CARTESIAN_POINT('Ctrl Pts',(-18.8163931962319,-21.0674335465806,
-4.51788920339165));
#76326=CARTESIAN_POINT('Ctrl Pts',(-18.8289813468477,-21.0669057385281,
-4.51863362607209));
#76327=CARTESIAN_POINT('Ctrl Pts',(-18.8900499132638,-21.0637988468246,
-4.52222991958248));
#76328=CARTESIAN_POINT('Ctrl Pts',(-18.9384387864532,-21.0596648830024,
-4.52503281529519));
#76329=CARTESIAN_POINT('Ctrl Pts',(-19.0271594313944,-21.0490006270932,
-4.53011167662205));
#76330=CARTESIAN_POINT('Ctrl Pts',(-19.0675252961146,-21.0429603546819,
-4.5323993561184));
#76331=CARTESIAN_POINT('Ctrl Pts',(-19.2400326012144,-21.0120235601538,
-4.54212611109203));
#76332=CARTESIAN_POINT('Ctrl Pts',(-19.3698061794308,-20.9757380922083,
-4.54929593551354));
#76333=CARTESIAN_POINT('Ctrl Pts',(-19.5537918917088,-20.9048350887584,
-4.56013222940999));
#76334=CARTESIAN_POINT('Ctrl Pts',(-19.6112871208758,-20.8796902727224,
-4.56362576714972));
#76335=CARTESIAN_POINT('Ctrl Pts',(-19.6953393038403,-20.8383914171856,
-4.56901248367176));
#76336=CARTESIAN_POINT('Ctrl Pts',(-19.7227978808744,-20.8241443212404,
-4.5708188659577));
#76337=CARTESIAN_POINT('Ctrl Pts',(-19.7561871501496,-20.8058805923223,
-4.57308543694436));
#76338=CARTESIAN_POINT('Ctrl Pts',(-19.7624240636873,-20.8024279943996,
-4.57351187890429));
#76339=CARTESIAN_POINT('Ctrl Pts',(-19.7722074770424,-20.7969474042102,
-4.57418582534221));
#76340=CARTESIAN_POINT('Ctrl Pts',(-19.7757658138193,-20.7949404977365,
-4.57443199751141));
#76341=CARTESIAN_POINT('Ctrl Pts',(-19.7824276977631,-20.7911577279672,
-4.57489489396021));
#76342=CARTESIAN_POINT('Ctrl Pts',(-19.7855325623306,-20.7893842971619,
-4.57511146199046));
#76343=CARTESIAN_POINT('Ctrl Pts',(-19.7926381815843,-20.7853018131917,
-4.57560897879283));
#76344=CARTESIAN_POINT('Ctrl Pts',(-19.7966358701506,-20.7829875325341,
-4.57589026235824));
#76345=CARTESIAN_POINT('Ctrl Pts',(-19.8089993459826,-20.7757761306816,
-4.57676436928368));
#76346=CARTESIAN_POINT('Ctrl Pts',(-19.8173389570027,-20.7708346996762,
-4.57735995760433));
#76347=CARTESIAN_POINT('Ctrl Pts',(-19.9078161053869,-20.7163816868856,
-4.58388436068923));
#76348=CARTESIAN_POINT('Ctrl Pts',(-19.986523198797,-20.661405824452,-4.59012233657905));
#76349=CARTESIAN_POINT('Ctrl Pts',(-20.1599400145677,-20.5218534134479,
-4.60477531850831));
#76350=CARTESIAN_POINT('Ctrl Pts',(-20.2513338677791,-20.4337041015626,
-4.61320515862001));
#76351=CARTESIAN_POINT('Ctrl Pts',(-20.3724500085333,-20.2938520750625,
-4.62512676308915));
#76352=CARTESIAN_POINT('Ctrl Pts',(-20.4087695858815,-20.2482381017544,
-4.62882513898398));
#76353=CARTESIAN_POINT('Ctrl Pts',(-20.4642421849682,-20.1723389341196,
-4.63467555352348));
#76354=CARTESIAN_POINT('Ctrl Pts',(-20.4845888313357,-20.142967724368,-4.63687127240738));
#76355=CARTESIAN_POINT('Ctrl Pts',(-20.5101992127512,-20.1039225947349,
-4.63970433693292));
#76356=CARTESIAN_POINT('Ctrl Pts',(-20.5161437266752,-20.0947042715433,
-4.64036713243605));
#76357=CARTESIAN_POINT('Ctrl Pts',(-20.5257284537054,-20.0795842397072,
-4.64144451610046));
#76358=CARTESIAN_POINT('Ctrl Pts',(-20.5294117352557,-20.0737101997125,
-4.6418607000435));
#76359=CARTESIAN_POINT('Ctrl Pts',(-20.5364622218308,-20.0623424943512,
-4.64266159601023));
#76360=CARTESIAN_POINT('Ctrl Pts',(-20.5398333285156,-20.0568513506027,
-4.643046449035));
#76361=CARTESIAN_POINT('Ctrl Pts',(-20.5475262599853,-20.0441911806493,
-4.64392917004843));
#76362=CARTESIAN_POINT('Ctrl Pts',(-20.5518307570477,-20.037011710788,-4.64442639942141));
#76363=CARTESIAN_POINT('Ctrl Pts',(-20.5632211405642,-20.0177556314884,
-4.64575121615546));
#76364=CARTESIAN_POINT('Ctrl Pts',(-20.5702300657121,-20.005633810653,-4.64657601092085));
#76365=CARTESIAN_POINT('Ctrl Pts',(-20.6269881215836,-19.9051849130035,
-4.6533376470631));
#76366=CARTESIAN_POINT('Ctrl Pts',(-20.6704575918116,-19.8134530243061,
-4.65904092207757));
#76367=CARTESIAN_POINT('Ctrl Pts',(-20.7124616914314,-19.7053857462978,
-4.66542611012426));
#76368=CARTESIAN_POINT('Ctrl Pts',(-20.7175920952023,-19.6917722147139,
-4.66622481928063));
#76369=CARTESIAN_POINT('Ctrl Pts',(-20.7225805678527,-19.6781104083805,
-4.66702139913379));
#76370=CARTESIAN_POINT('',(-20.8509999970068,-18.9521080404548,-3.68920542733227));
#76371=CARTESIAN_POINT('Ctrl Pts',(-20.7225805839746,-19.678110364228,-4.44630500845845));
#76372=CARTESIAN_POINT('Ctrl Pts',(-20.7059750529334,-19.7235875234065,
-4.44325060284348));
#76373=CARTESIAN_POINT('Ctrl Pts',(-20.6878139586179,-19.7684827791584,
-4.4401292757464));
#76374=CARTESIAN_POINT('Ctrl Pts',(-20.591907891162,-19.983994763893,-4.42474709701318));
#76375=CARTESIAN_POINT('Ctrl Pts',(-20.4932541629939,-20.1444257471549,
-4.41214843505669));
#76376=CARTESIAN_POINT('Ctrl Pts',(-20.3393458867707,-20.3331927496265,
-4.39674509708733));
#76377=CARTESIAN_POINT('Ctrl Pts',(-20.3022244749473,-20.3752012331731,
-4.39326454066552));
#76378=CARTESIAN_POINT('Ctrl Pts',(-20.2551575499931,-20.42438360834,-4.38912061286533));
#76379=CARTESIAN_POINT('Ctrl Pts',(-20.2467641763983,-20.4330058534641,
-4.38839137665417));
#76380=CARTESIAN_POINT('Ctrl Pts',(-20.2327633547897,-20.4471452342441,
-4.38719077628363));
#76381=CARTESIAN_POINT('Ctrl Pts',(-20.2271979391164,-20.4527034291847,
-4.38671758281733));
#76382=CARTESIAN_POINT('Ctrl Pts',(-20.2170712572065,-20.4627048652255,
-4.38586381042063));
#76383=CARTESIAN_POINT('Ctrl Pts',(-20.2125206967677,-20.4671587687003,
-4.3854827629929));
#76384=CARTESIAN_POINT('Ctrl Pts',(-20.2027146609815,-20.4766702731645,
-4.38466716985252));
#76385=CARTESIAN_POINT('Ctrl Pts',(-20.1974529921072,-20.4817213926687,
-4.3842329096807));
#76386=CARTESIAN_POINT('Ctrl Pts',(-20.1830322987544,-20.4954225290718,
-4.38305178219053));
#76387=CARTESIAN_POINT('Ctrl Pts',(-20.1738219073444,-20.5040182317033,
-4.38230725975863));
#76388=CARTESIAN_POINT('Ctrl Pts',(-20.1246867769961,-20.5490602827635,
-4.378386182477));
#76389=CARTESIAN_POINT('Ctrl Pts',(-20.0834517180678,-20.584051482861,-4.3752714719419));
#76390=CARTESIAN_POINT('Ctrl Pts',(-19.8904571533231,-20.7355010553542,
-4.36137514659493));
#76391=CARTESIAN_POINT('Ctrl Pts',(-19.7247036441514,-20.8326301520677,
-4.3513510585107));
#76392=CARTESIAN_POINT('Ctrl Pts',(-19.5328945419942,-20.9125433624371,
-4.33980005282473));
#76393=CARTESIAN_POINT('Ctrl Pts',(-19.5175474424909,-20.9187272689795,
-4.33887548281398));
#76394=CARTESIAN_POINT('Ctrl Pts',(-19.452565118001,-20.9440296882608,-4.33495319392707));
#76395=CARTESIAN_POINT('Ctrl Pts',(-19.4022951099149,-20.9614523489393,
-4.33190077680262));
#76396=CARTESIAN_POINT('Ctrl Pts',(-19.3430953186911,-20.9795028405317,
-4.32822794047945));
#76397=CARTESIAN_POINT('Ctrl Pts',(-19.3347479195817,-20.981991824327,-4.32770827127453));
#76398=CARTESIAN_POINT('Ctrl Pts',(-19.3220834068493,-20.9856831089112,
-4.32691680809558));
#76399=CARTESIAN_POINT('Ctrl Pts',(-19.3177773277268,-20.9869233675167,
-4.32664717278153));
#76400=CARTESIAN_POINT('Ctrl Pts',(-19.3100396533694,-20.989125430285,-4.32616165788158));
#76401=CARTESIAN_POINT('Ctrl Pts',(-19.3066095412356,-20.9900922486373,
-4.32594607368808));
#76402=CARTESIAN_POINT('Ctrl Pts',(-19.2991494694688,-20.9921746400132,
-4.32547642114468));
#76403=CARTESIAN_POINT('Ctrl Pts',(-19.295118693786,-20.9932869213757,-4.32522217096642));
#76404=CARTESIAN_POINT('Ctrl Pts',(-19.2837834444003,-20.9963787414552,
-4.32450584948313));
#76405=CARTESIAN_POINT('Ctrl Pts',(-19.2764716985071,-20.998331040325,-4.32404224614419));
#76406=CARTESIAN_POINT('Ctrl Pts',(-19.232618159204,-21.0097887625457,-4.32125312336358));
#76407=CARTESIAN_POINT('Ctrl Pts',(-19.1958402651079,-21.0183537503357,
-4.31887850060007));
#76408=CARTESIAN_POINT('Ctrl Pts',(-19.0738755684451,-21.0433388780075,
-4.31093035876734));
#76409=CARTESIAN_POINT('Ctrl Pts',(-18.9879109198764,-21.0555068432524,
-4.30521476113107));
#76410=CARTESIAN_POINT('Ctrl Pts',(-18.7261811852056,-21.0762739786108,
-4.28786797528356));
#76411=CARTESIAN_POINT('Ctrl Pts',(-18.5498271357661,-21.0682951159875,
-4.27632332416896));
#76412=CARTESIAN_POINT('Ctrl Pts',(-18.3538341836113,-21.0347122447921,
-4.26408410894484));
#76413=CARTESIAN_POINT('Ctrl Pts',(-18.3312640457341,-21.0304658185513,
-4.26268226389162));
#76414=CARTESIAN_POINT('Ctrl Pts',(-18.299419550179,-21.0239362625587,-4.26071447593337));
#76415=CARTESIAN_POINT('Ctrl Pts',(-18.2900852985823,-21.0219564695907,
-4.26013890950837));
#76416=CARTESIAN_POINT('Ctrl Pts',(-18.274936970614,-21.0186363318461,-4.25920675779561));
#76417=CARTESIAN_POINT('Ctrl Pts',(-18.2691146907666,-21.0173344144343,
-4.25884894658992));
#76418=CARTESIAN_POINT('Ctrl Pts',(-18.2569360706598,-21.0145570502935,
-4.25810144260337));
#76419=CARTESIAN_POINT('Ctrl Pts',(-18.2505808835106,-21.0130767908245,
-4.25771190874602));
#76420=CARTESIAN_POINT('Ctrl Pts',(-18.2354732802992,-21.0094841855936,
-4.2567871363927));
#76421=CARTESIAN_POINT('Ctrl Pts',(-18.2267272505224,-21.0073453300298,
-4.25625275703224));
#76422=CARTESIAN_POINT('Ctrl Pts',(-18.1972843532456,-20.999945638784,-4.2544569315623));
#76423=CARTESIAN_POINT('Ctrl Pts',(-18.1766530921176,-20.9944273544678,
-4.25320379655168));
#76424=CARTESIAN_POINT('Ctrl Pts',(-18.0646403429302,-20.9626433453724,
-4.24642355657773));
#76425=CARTESIAN_POINT('Ctrl Pts',(-17.9750191843356,-20.930555075165,-4.24109076819345));
#76426=CARTESIAN_POINT('Ctrl Pts',(-17.7316760138036,-20.8244484976068,
-4.22648574375833));
#76427=CARTESIAN_POINT('Ctrl Pts',(-17.5843122092003,-20.7377555286927,
-4.2175229278678));
#76428=CARTESIAN_POINT('Ctrl Pts',(-17.4194338798366,-20.6118144254466,
-4.20567685724372));
#76429=CARTESIAN_POINT('Ctrl Pts',(-17.3905232962856,-20.5885017510247,
-4.20352037051548));
#76430=CARTESIAN_POINT('Ctrl Pts',(-17.3567868496268,-20.5598010600513,
-4.20088718598271));
#76431=CARTESIAN_POINT('Ctrl Pts',(-17.3513546411945,-20.5551319717157,
-4.20045946944414));
#76432=CARTESIAN_POINT('Ctrl Pts',(-17.3425343964042,-20.5474726239438,
-4.19975869027246));
#76433=CARTESIAN_POINT('Ctrl Pts',(-17.3391320035622,-20.5444988826961,
-4.19948682220336));
#76434=CARTESIAN_POINT('Ctrl Pts',(-17.3330613329158,-20.539158647118,-4.19899892069522));
#76435=CARTESIAN_POINT('Ctrl Pts',(-17.3303894915829,-20.5367962835783,
-4.19878319535851));
#76436=CARTESIAN_POINT('Ctrl Pts',(-17.3246190913873,-20.5316682259454,
-4.19831513323318));
#76437=CARTESIAN_POINT('Ctrl Pts',(-17.3215227405428,-20.5289001999034,
-4.19806262490934));
#76438=CARTESIAN_POINT('Ctrl Pts',(-17.3129036055194,-20.5211492499445,
-4.19735600543973));
#76439=CARTESIAN_POINT('Ctrl Pts',(-17.3073989722264,-20.5161463597715,
-4.19690042684133));
#76440=CARTESIAN_POINT('Ctrl Pts',(-17.2757206373601,-20.487049153316,-4.19425429279777));
#76441=CARTESIAN_POINT('Ctrl Pts',(-17.2501328775237,-20.4623286462916,
-4.19202019468405));
#76442=CARTESIAN_POINT('Ctrl Pts',(-17.1701409974656,-20.3810525079773,
-4.18475370112295));
#76443=CARTESIAN_POINT('Ctrl Pts',(-17.1182555550447,-20.3221146949031,
-4.17960301470105));
#76444=CARTESIAN_POINT('Ctrl Pts',(-16.9534976510358,-20.1125549463459,
-4.16200818529868));
#76445=CARTESIAN_POINT('Ctrl Pts',(-16.8574333061634,-19.9497988824915,
-4.14960212188181));
#76446=CARTESIAN_POINT('Ctrl Pts',(-16.7756363194314,-19.7563492369065,
-4.13668902326418));
#76447=CARTESIAN_POINT('Ctrl Pts',(-16.7674421701439,-19.7361022625955,
-4.13535674821671));
#76448=CARTESIAN_POINT('Ctrl Pts',(-16.7565261363091,-19.7078815777027,
-4.1335256874127));
#76449=CARTESIAN_POINT('Ctrl Pts',(-16.753536519592,-19.7000135340097,-4.13301793609186));
#76450=CARTESIAN_POINT('Ctrl Pts',(-16.7484728288283,-19.686443775432,-4.13214690571609));
#76451=CARTESIAN_POINT('Ctrl Pts',(-16.746376212341,-19.6807506340686,-4.1317828754104));
#76452=CARTESIAN_POINT('Ctrl Pts',(-16.7420994336397,-19.6689817292357,
-4.13103321838409));
#76453=CARTESIAN_POINT('Ctrl Pts',(-16.7399225263875,-19.6629048438291,
-4.13064770341623));
#76454=CARTESIAN_POINT('Ctrl Pts',(-16.7349131486048,-19.6487169933402,
-4.12975124249218));
#76455=CARTESIAN_POINT('Ctrl Pts',(-16.7321021768789,-19.6405985167946,
-4.12924101486907));
#76456=CARTESIAN_POINT('Ctrl Pts',(-16.7232307638172,-19.6144631363991,
-4.12760708048881));
#76457=CARTESIAN_POINT('Ctrl Pts',(-16.7173634250955,-19.5963813217992,
-4.12648974845712));
#76458=CARTESIAN_POINT('Ctrl Pts',(-16.6891028975398,-19.5051196249743,
-4.12091263309419));
#76459=CARTESIAN_POINT('Ctrl Pts',(-16.6704446171377,-19.4308386516401,
-4.11657589146647));
#76460=CARTESIAN_POINT('Ctrl Pts',(-16.6348945456058,-19.2478371293008,
-4.10621551847124));
#76461=CARTESIAN_POINT('Ctrl Pts',(-16.6223700923974,-19.1385027329552,
-4.10030128258774));
#76462=CARTESIAN_POINT('Ctrl Pts',(-16.6158499422204,-18.9586296005015,
-4.09049861521862));
#76463=CARTESIAN_POINT('Ctrl Pts',(-16.6167921119604,-18.8884923012791,
-4.08665523106028));
#76464=CARTESIAN_POINT('Ctrl Pts',(-16.6242519040962,-18.7704011489976,
-4.07997133316755));
#76465=CARTESIAN_POINT('Ctrl Pts',(-16.6289363433943,-18.7223885939147,
-4.07719364272327));
#76466=CARTESIAN_POINT('Ctrl Pts',(-16.6362711963348,-18.6668983742835,
-4.07387055095543));
#76467=CARTESIAN_POINT('Ctrl Pts',(-16.6373290194225,-18.6592204485359,
-4.07340822687095));
#76468=CARTESIAN_POINT('Ctrl Pts',(-16.6390882420684,-18.6469503226795,
-4.07266509892751));
#76469=CARTESIAN_POINT('Ctrl Pts',(-16.6397626491681,-18.6423542401508,
-4.07238577830725));
#76470=CARTESIAN_POINT('Ctrl Pts',(-16.6409847634691,-18.6342121878138,
-4.07188918875754));
#76471=CARTESIAN_POINT('Ctrl Pts',(-16.6415263646599,-18.6306653470811,
-4.07167226758135));
#76472=CARTESIAN_POINT('Ctrl Pts',(-16.6426944554599,-18.6231439395748,
-4.0712109783146));
#76473=CARTESIAN_POINT('Ctrl Pts',(-16.6433232501197,-18.6191698391243,
-4.07096648742731));
#76474=CARTESIAN_POINT('Ctrl Pts',(-16.6450531811568,-18.608434704283,-4.07030404437638));
#76475=CARTESIAN_POINT('Ctrl Pts',(-16.6461757994061,-18.6016772504882,
-4.06988490316812));
#76476=CARTESIAN_POINT('Ctrl Pts',(-16.651940782872,-18.5679878934548,-4.06778492686652));
#76477=CARTESIAN_POINT('Ctrl Pts',(-16.6570713312078,-18.5411435506829,
-4.06607862011139));
#76478=CARTESIAN_POINT('Ctrl Pts',(-16.6734618060952,-18.4635616165769,
-4.0610657501009));
#76479=CARTESIAN_POINT('Ctrl Pts',(-16.6860717907079,-18.4131317184198,
-4.05770556997723));
#76480=CARTESIAN_POINT('Ctrl Pts',(-16.7391454266503,-18.2298304943454,
-4.04523014415083));
#76481=CARTESIAN_POINT('Ctrl Pts',(-16.7908028922377,-18.1005525454839,
-4.03594380839722));
#76482=CARTESIAN_POINT('Ctrl Pts',(-16.898623103787,-17.8926792547821,-4.02078720699884));
#76483=CARTESIAN_POINT('Ctrl Pts',(-16.9481619569181,-17.8111425896993,
-4.01476927491229));
#76484=CARTESIAN_POINT('Ctrl Pts',(-17.0110098080695,-17.7218838531483,
-4.00810746113588));
#76485=CARTESIAN_POINT('Ctrl Pts',(-17.019096971541,-17.7106343997278,-4.00726627211872));
#76486=CARTESIAN_POINT('Ctrl Pts',(-17.0322212446878,-17.6927512486061,
-4.00592627440369));
#76487=CARTESIAN_POINT('Ctrl Pts',(-17.0371879774477,-17.6860666237372,
-4.0054247607819));
#76488=CARTESIAN_POINT('Ctrl Pts',(-17.0460632962751,-17.6742675890925,
-4.00453835475868));
#76489=CARTESIAN_POINT('Ctrl Pts',(-17.0499559830554,-17.6691414029297,
-4.00415284763788));
#76490=CARTESIAN_POINT('Ctrl Pts',(-17.058101743891,-17.6585154158186,-4.00335286100862));
#76491=CARTESIAN_POINT('Ctrl Pts',(-17.0623586579445,-17.6530186453811,
-4.00293853933194));
#76492=CARTESIAN_POINT('Ctrl Pts',(-17.073454498603,-17.6388359391721,-4.00186816347282));
#76493=CARTESIAN_POINT('Ctrl Pts',(-17.0803345773694,-17.6301823537766,
-4.00121375332688));
#76494=CARTESIAN_POINT('Ctrl Pts',(-17.1102289631788,-17.5931807114727,
-3.99840935811378));
#76495=CARTESIAN_POINT('Ctrl Pts',(-17.1339075922544,-17.5653757678634,
-3.99628627007465));
#76496=CARTESIAN_POINT('Ctrl Pts',(-17.1984212854729,-17.4934743137192,
-3.99073907288807));
#76497=CARTESIAN_POINT('Ctrl Pts',(-17.2404354309439,-17.4504791556932,
-3.98736295770136));
#76498=CARTESIAN_POINT('Ctrl Pts',(-17.4057125679295,-17.2951547469706,
-3.97480002707343));
#76499=CARTESIAN_POINT('Ctrl Pts',(-17.5402502319539,-17.1957432471182,
-3.96602173154569));
#76500=CARTESIAN_POINT('Ctrl Pts',(-17.7323969635959,-17.0861349624229,
-3.95359315730816));
#76501=CARTESIAN_POINT('Ctrl Pts',(-17.7807716781396,-17.0609643930868,
-3.95046757089726));
#76502=CARTESIAN_POINT('Ctrl Pts',(-17.83798496002,-17.0339481559771,-3.94671321259899));
#76503=CARTESIAN_POINT('Ctrl Pts',(-17.8459339283735,-17.0302548361845,
-3.94619033276576));
#76504=CARTESIAN_POINT('Ctrl Pts',(-17.857991688379,-17.0247432386701,-3.94539493128373));
#76505=CARTESIAN_POINT('Ctrl Pts',(-17.8620838225065,-17.0228884519835,
-3.94512460056052));
#76506=CARTESIAN_POINT('Ctrl Pts',(-17.8694331455228,-17.019585484245,-3.94463834535009));
#76507=CARTESIAN_POINT('Ctrl Pts',(-17.872688113209,-17.018132491626,-3.94442272021774));
#76508=CARTESIAN_POINT('Ctrl Pts',(-17.8797611811931,-17.0149965280794,
-3.94395357670426));
#76509=CARTESIAN_POINT('Ctrl Pts',(-17.8835805411395,-17.0133166444499,
-3.94369987975458));
#76510=CARTESIAN_POINT('Ctrl Pts',(-17.8943035217731,-17.0086380993906,
-3.94298664442694));
#76511=CARTESIAN_POINT('Ctrl Pts',(-17.9012181245005,-17.0056649835608,
-3.94252559469452));
#76512=CARTESIAN_POINT('Ctrl Pts',(-17.9422593749615,-16.9882769531812,
-3.93978303617392));
#76513=CARTESIAN_POINT('Ctrl Pts',(-17.9767415780873,-16.9747239147111,
-3.93745427279839));
#76514=CARTESIAN_POINT('Ctrl Pts',(-18.0904942376852,-16.9334259096005,
-3.92973304932975));
#76515=CARTESIAN_POINT('Ctrl Pts',(-18.1710597367467,-16.9094923620726,
-3.92420662595751));
#76516=CARTESIAN_POINT('Ctrl Pts',(-18.4279500089406,-16.8495345638189,
-3.90678197133828));
#76517=CARTESIAN_POINT('Ctrl Pts',(-18.6076051857285,-16.8311329485589,
-3.89495694896189));
#76518=CARTESIAN_POINT('Ctrl Pts',(-18.8100807322765,-16.8362463906006,
-3.88249451686865));
#76519=CARTESIAN_POINT('Ctrl Pts',(-18.8327045134775,-16.8371810727607,
-3.88111267460419));
#76520=CARTESIAN_POINT('Ctrl Pts',(-18.8647825400151,-16.8390222532311,
-3.87916783765606));
#76521=CARTESIAN_POINT('Ctrl Pts',(-18.8742517772229,-16.8396296549411,
-3.87859552139535));
#76522=CARTESIAN_POINT('Ctrl Pts',(-18.889658208021,-16.840721950844,-3.87766719336879));
#76523=CARTESIAN_POINT('Ctrl Pts',(-18.8955979253899,-16.8411682705131,
-3.87730997557107));
#76524=CARTESIAN_POINT('Ctrl Pts',(-18.9080490546663,-16.8421567315635,
-3.87656256512833));
#76525=CARTESIAN_POINT('Ctrl Pts',(-18.9145600085186,-16.8427039620772,
-3.87617253644228));
#76526=CARTESIAN_POINT('Ctrl Pts',(-18.9300836147993,-16.8440810902564,
-3.87524449652174));
#76527=CARTESIAN_POINT('Ctrl Pts',(-18.9390937311685,-16.8449386626497,
-3.874707360787));
#76528=CARTESIAN_POINT('Ctrl Pts',(-18.9696216472435,-16.8480419476245,
-3.87289236579694));
#76529=CARTESIAN_POINT('Ctrl Pts',(-18.9911108687225,-16.8505597560181,
-3.87162306511117));
#76530=CARTESIAN_POINT('Ctrl Pts',(-19.1091483882639,-16.8662275521552,
-3.86469120335776));
#76531=CARTESIAN_POINT('Ctrl Pts',(-19.2047439228792,-16.8857022471294,
-3.85923328847979));
#76532=CARTESIAN_POINT('Ctrl Pts',(-19.4494677928498,-16.9534311374556,
-3.84527878745208));
#76533=CARTESIAN_POINT('Ctrl Pts',(-19.5951621838004,-17.0117516735864,
-3.8370068749821));
#76534=CARTESIAN_POINT('Ctrl Pts',(-19.774743453748,-17.107881141832,-3.82549065724233));
#76535=CARTESIAN_POINT('Ctrl Pts',(-19.8156366621528,-17.1315652447075,
-3.82276760727552));
#76536=CARTESIAN_POINT('Ctrl Pts',(-19.8627994039801,-17.1610307145722,
-3.81946565200369));
#76537=CARTESIAN_POINT('Ctrl Pts',(-19.8698723625714,-17.1655081734109,
-3.81896606295435));
#76538=CARTESIAN_POINT('Ctrl Pts',(-19.880586834266,-17.1723802023097,-3.81820225254096));
#76539=CARTESIAN_POINT('Ctrl Pts',(-19.8842479096312,-17.1747443238376,
-3.81794000883896));
#76540=CARTESIAN_POINT('Ctrl Pts',(-19.8907254749626,-17.1789555786331,
-3.81747374310823));
#76541=CARTESIAN_POINT('Ctrl Pts',(-19.893544881643,-17.1807981448131,-3.81727002725082));
#76542=CARTESIAN_POINT('Ctrl Pts',(-19.8963810206393,-17.1826613202964,
-3.81706431919753));
#76543=CARTESIAN_POINT('Ctrl Pts',(-19.8964021259494,-17.1826751857768,
-3.81706278836429));
#76544=CARTESIAN_POINT('Ctrl Pts',(-19.8964439371482,-17.1827026554021,
-3.81705975558274));
#76545=CARTESIAN_POINT('Ctrl Pts',(-19.8964646431052,-17.1827162595717,
-3.81705825363111));
#76546=CARTESIAN_POINT('Ctrl Pts',(-19.8965056793506,-17.1827432221214,
-3.81705527689466));
#76547=CARTESIAN_POINT('Ctrl Pts',(-19.8965260095775,-17.1827565804425,
-3.81705380211581));
#76548=CARTESIAN_POINT('Ctrl Pts',(-19.8965663163984,-17.1827830657188,
-3.8170508781309));
#76549=CARTESIAN_POINT('Ctrl Pts',(-19.896586292861,-17.1827961925705,-3.81704942893576));
#76550=CARTESIAN_POINT('Ctrl Pts',(-19.8966259124454,-17.182822228191,-3.81704655465032));
#76551=CARTESIAN_POINT('Ctrl Pts',(-19.8966455555369,-17.182835136924,-3.81704512956349));
#76552=CARTESIAN_POINT('Ctrl Pts',(-19.8966845271922,-17.182860748623,-3.81704230213364));
#76553=CARTESIAN_POINT('Ctrl Pts',(-19.8967038558692,-17.1828734516486,
-3.81704089978359));
#76554=CARTESIAN_POINT('Ctrl Pts',(-19.8967422163445,-17.1828986634879,
-3.81703811655034));
#76555=CARTESIAN_POINT('Ctrl Pts',(-19.8967612482861,-17.182911172382,-3.81703673565787));
#76556=CARTESIAN_POINT('Ctrl Pts',(-19.8967990320516,-17.1829360069337,
-3.81703399412695));
#76557=CARTESIAN_POINT('Ctrl Pts',(-19.8968177838715,-17.182948332576,-3.81703263348984));
#76558=CARTESIAN_POINT('Ctrl Pts',(-19.896855023109,-17.1829728109156,-3.8170299313324));
#76559=CARTESIAN_POINT('Ctrl Pts',(-19.8968735104283,-17.1829849635366,
-3.81702858982017));
#76560=CARTESIAN_POINT('Ctrl Pts',(-19.8969102351793,-17.1830091053395,
-3.81702592486214));
#76561=CARTESIAN_POINT('Ctrl Pts',(-19.8969284726153,-17.1830210945133,
-3.81702460141691));
#76562=CARTESIAN_POINT('Ctrl Pts',(-19.8969647110558,-17.1830449182348,
-3.81702197161905));
#76563=CARTESIAN_POINT('Ctrl Pts',(-19.8969827122019,-17.1830567528652,
-3.81702066525698));
#76564=CARTESIAN_POINT('Ctrl Pts',(-19.8970184914677,-17.1830802762825,
-3.8170180686551));
#76565=CARTESIAN_POINT('Ctrl Pts',(-19.8970362694361,-17.1830919649601,
-3.81701677842706));
#76566=CARTESIAN_POINT('Ctrl Pts',(-19.8970716142431,-17.1831152042646,
-3.81701421323215));
#76567=CARTESIAN_POINT('Ctrl Pts',(-19.8970891811503,-17.1831267549276,
-3.81701293826105));
#76568=CARTESIAN_POINT('Ctrl Pts',(-19.8971241154634,-17.183149725822,-3.81701040273822));
#76569=CARTESIAN_POINT('Ctrl Pts',(-19.897141482875,-17.1831611460488,-3.81700914218676));
#76570=CARTESIAN_POINT('Ctrl Pts',(-19.8971760290475,-17.1831838631808,
-3.81700663471771));
#76571=CARTESIAN_POINT('Ctrl Pts',(-19.8971932078295,-17.1831951600919,
-3.81700538779921));
#76572=CARTESIAN_POINT('Ctrl Pts',(-19.897227387305,-17.1832176375151,-3.81700290683131));
#76573=CARTESIAN_POINT('Ctrl Pts',(-19.8972443878677,-17.1832288179337,
-3.817001672792));
#76574=CARTESIAN_POINT('Ctrl Pts',(-19.8972782207694,-17.1832510688373,
-3.81699921686815));
#76575=CARTESIAN_POINT('Ctrl Pts',(-19.8972950529995,-17.1832621392437,
-3.81699799499209));
#76576=CARTESIAN_POINT('Ctrl Pts',(-19.8973285583645,-17.1832841761064,
-3.81699556273376));
#76577=CARTESIAN_POINT('Ctrl Pts',(-19.897345231592,-17.183295142617,-3.8169943523453));
#76578=CARTESIAN_POINT('Ctrl Pts',(-19.8973784275216,-17.1833169773053,
-3.81699194244158));
#76579=CARTESIAN_POINT('Ctrl Pts',(-19.8973949504846,-17.1833278456486,
-3.81699074290788));
#76580=CARTESIAN_POINT('Ctrl Pts',(-19.8974278547195,-17.1833494897954,
-3.8169883540738));
#76581=CARTESIAN_POINT('Ctrl Pts',(-19.8974442359604,-17.1833602655727,
-3.81698716477612));
#76582=CARTESIAN_POINT('Ctrl Pts',(-19.8974768649881,-17.1833817299893,
-3.81698479581742));
#76583=CARTESIAN_POINT('Ctrl Pts',(-19.8974931126518,-17.1833924185422,
-3.81698361616577));
#76584=CARTESIAN_POINT('Ctrl Pts',(-19.90101725197,-17.1857108491017,-3.81672774259221));
#76585=CARTESIAN_POINT('Ctrl Pts',(-19.9045182350899,-17.1880289992199,
-3.81647234691026));
#76586=CARTESIAN_POINT('Ctrl Pts',(-19.9146081885047,-17.1947532518542,
-3.81573286041144));
#76587=CARTESIAN_POINT('Ctrl Pts',(-19.9211792553152,-17.1991859083652,
-3.81524703302925));
#76588=CARTESIAN_POINT('Ctrl Pts',(-19.9646746055134,-17.2288834234257,
-3.81200380529768));
#76589=CARTESIAN_POINT('Ctrl Pts',(-20.0008121180661,-17.2552745868262,
-3.80917735043901));
#76590=CARTESIAN_POINT('Ctrl Pts',(-20.1294156491835,-17.3555929152385,
-3.79870576291934));
#76591=CARTESIAN_POINT('Ctrl Pts',(-20.216473553393,-17.4360940750762,-3.79081709998143));
#76592=CARTESIAN_POINT('Ctrl Pts',(-20.3960790574005,-17.6325203492072,
-3.77328192696135));
#76593=CARTESIAN_POINT('Ctrl Pts',(-20.4841331800545,-17.7517573356269,
-3.76375301034587));
#76594=CARTESIAN_POINT('Ctrl Pts',(-20.5662675611358,-17.891487325838,-3.75385703836535));
#76595=CARTESIAN_POINT('Ctrl Pts',(-20.5733557627424,-17.9038292404177,
-3.75299259719209));
#76596=CARTESIAN_POINT('Ctrl Pts',(-20.5844473891295,-17.9236009249835,
-3.75162281076882));
#76597=CARTESIAN_POINT('Ctrl Pts',(-20.5885316858317,-17.9309846098627,
-3.75111456735481));
#76598=CARTESIAN_POINT('Ctrl Pts',(-20.5956619115805,-17.9440587412643,
-3.75022037175344));
#76599=CARTESIAN_POINT('Ctrl Pts',(-20.5987261475108,-17.9497390308349,
-3.74983376889326));
#76600=CARTESIAN_POINT('Ctrl Pts',(-20.6050148169184,-17.9615252491383,
-3.74903547104967));
#76601=CARTESIAN_POINT('Ctrl Pts',(-20.6082354533443,-17.9676331251069,
-3.74862391431566));
#76602=CARTESIAN_POINT('Ctrl Pts',(-20.6164350746077,-17.9833696844013,
-3.74756898125616));
#76603=CARTESIAN_POINT('Ctrl Pts',(-20.621370133545,-17.9930211243061,-3.74692715903245));
#76604=CARTESIAN_POINT('Ctrl Pts',(-20.6417352834016,-18.0336152246479,
-3.74424881006918));
#76605=CARTESIAN_POINT('Ctrl Pts',(-20.6564807857285,-18.064896659469,-3.74223621312865));
#76606=CARTESIAN_POINT('Ctrl Pts',(-20.6929644865468,-18.1474813595387,
-3.73704320781428));
#76607=CARTESIAN_POINT('Ctrl Pts',(-20.7134559977444,-18.1993070222144,
-3.73390317844735));
#76608=CARTESIAN_POINT('Ctrl Pts',(-20.7653540629842,-18.3474054561233,
-3.72518160212191));
#76609=CARTESIAN_POINT('Ctrl Pts',(-20.7919349482263,-18.4452075808195,
-3.71971762169302));
#76610=CARTESIAN_POINT('Ctrl Pts',(-20.8347036733654,-18.6632602447623,
-3.70763489487761));
#76611=CARTESIAN_POINT('Ctrl Pts',(-20.847766551041,-18.7837459212227,-3.70102041173113));
#76612=CARTESIAN_POINT('Ctrl Pts',(-20.850728113419,-18.9161735210989,-3.69321415810316));
#76613=CARTESIAN_POINT('Ctrl Pts',(-20.8508915887521,-18.9276806435142,
-3.69253136286732));
#76614=CARTESIAN_POINT('Ctrl Pts',(-20.8509827903195,-18.9427504062806,
-3.69163064214214));
#76615=CARTESIAN_POINT('Ctrl Pts',(-20.8509953572148,-18.9463125920937,
-3.69141725226841));
#76616=CARTESIAN_POINT('Ctrl Pts',(-20.850999717921,-18.9506563959296,-3.69115643925956));
#76617=CARTESIAN_POINT('Ctrl Pts',(-20.8510000697051,-18.9514380271121,
-3.69110948441178));
#76618=CARTESIAN_POINT('Ctrl Pts',(-20.8509999886044,-18.9522196567131,
-3.69106250577301));
#76619=CARTESIAN_POINT('Ctrl Pts',(-20.8509999976816,-18.952099076172,-3.6890562790225));
#76620=CARTESIAN_POINT('Ctrl Pts',(-20.8509997507685,-18.9573749670545,
-3.68873698393553));
#76621=CARTESIAN_POINT('Ctrl Pts',(-20.8509797813958,-18.9626508039048,
-3.68841768884856));
#76622=CARTESIAN_POINT('Ctrl Pts',(-20.8509400905189,-18.9679264921966,
-3.68809839376159));
#76623=CARTESIAN_POINT('Ctrl Pts',(-20.8503947174663,-19.0404171615265,
-3.68371111511894));
#76624=CARTESIAN_POINT('Ctrl Pts',(-20.8461205125485,-19.1130212561315,
-3.67932383647628));
#76625=CARTESIAN_POINT('Ctrl Pts',(-20.8381029246827,-19.1853235571938,
-3.67493655783363));
#76626=CARTESIAN_POINT('Ctrl Pts',(-20.8300957679123,-19.257531791037,-3.67055498715732));
#76627=CARTESIAN_POINT('Ctrl Pts',(-20.8183549391221,-19.3294385348818,
-3.66617341648101));
#76628=CARTESIAN_POINT('Ctrl Pts',(-20.8029178766228,-19.4006288218456,
-3.6617918458047));
#76629=CARTESIAN_POINT('Ctrl Pts',(-20.7874985864907,-19.4717371489208,
-3.65741531953908));
#76630=CARTESIAN_POINT('Ctrl Pts',(-20.7683916165406,-19.542130188401,-3.65303879327345));
#76631=CARTESIAN_POINT('Ctrl Pts',(-20.7456859385557,-19.6114002461458,
-3.64866226700783));
#76632=CARTESIAN_POINT('Ctrl Pts',(-20.7383572889959,-19.6337583531595,
-3.64724966759936));
#76633=CARTESIAN_POINT('Ctrl Pts',(-20.730654129157,-19.6559995449129,-3.64583706819089));
#76634=CARTESIAN_POINT('Ctrl Pts',(-20.7225805821191,-19.6781103693095,
-3.64442446878243));
#76635=CARTESIAN_POINT('Origin',(-18.734,-18.952,0.));
#76636=CARTESIAN_POINT('',(-20.7202230519095,-19.6772708889146,-2.84456322442383));
#76637=CARTESIAN_POINT('',(-20.7225805657411,-19.6781104141636,-3.06515450115675));
#76638=CARTESIAN_POINT('',(-20.7225805821191,-19.6781103693095,0.));
#76639=CARTESIAN_POINT('Ctrl Pts',(-20.7225805657411,-19.6781104141636,
-3.06515450115675));
#76640=CARTESIAN_POINT('Ctrl Pts',(-20.7750121871659,-19.5345172341707,
-3.0751267565293));
#76641=CARTESIAN_POINT('Ctrl Pts',(-20.8117530434534,-19.3856243798708,
-3.08537389662126));
#76642=CARTESIAN_POINT('Ctrl Pts',(-20.8399080668057,-19.17616159463,-3.09899381870072));
#76643=CARTESIAN_POINT('Ctrl Pts',(-20.8452891027995,-19.1180014933404,
-3.10269885507837));
#76644=CARTESIAN_POINT('Ctrl Pts',(-20.8500786753983,-19.0239677445121,
-3.10855854633529));
#76645=CARTESIAN_POINT('Ctrl Pts',(-20.8509926290102,-18.9882045641041,
-3.11075705378731));
#76646=CARTESIAN_POINT('Ctrl Pts',(-20.8510022031607,-18.9414601962185,
-3.11359314044188));
#76647=CARTESIAN_POINT('Ctrl Pts',(-20.8509191302795,-18.9304867805795,
-3.11425623710019));
#76648=CARTESIAN_POINT('Ctrl Pts',(-20.8506443291055,-18.9125808604659,
-3.11533398638087));
#76649=CARTESIAN_POINT('Ctrl Pts',(-20.8505038547663,-18.9056478799212,
-3.11575023684162));
#76650=CARTESIAN_POINT('Ctrl Pts',(-20.8501671510856,-18.8922748000332,
-3.11655117669939));
#76651=CARTESIAN_POINT('Ctrl Pts',(-20.8499755814641,-18.8858346698847,
-3.11693600754339));
#76652=CARTESIAN_POINT('Ctrl Pts',(-20.8494626513867,-18.8708874756035,
-3.1178271791705));
#76653=CARTESIAN_POINT('Ctrl Pts',(-20.8491193705504,-18.8623812375752,
-3.11833282785324));
#76654=CARTESIAN_POINT('Ctrl Pts',(-20.8478634332364,-18.835313502854,-3.11993722523715));
#76655=CARTESIAN_POINT('Ctrl Pts',(-20.8467576626712,-18.8167615275721,
-3.12102992330274));
#76656=CARTESIAN_POINT('Ctrl Pts',(-20.8436139259455,-18.7735961489326,
-3.12355760465782));
#76657=CARTESIAN_POINT('Ctrl Pts',(-20.8413892485388,-18.7489988246942,
-3.12498678499905));
#76658=CARTESIAN_POINT('Ctrl Pts',(-20.8320826356473,-18.6629186365409,
-3.12995537998052));
#76659=CARTESIAN_POINT('Ctrl Pts',(-20.8227356958111,-18.6017103544863,
-3.13342821369199));
#76660=CARTESIAN_POINT('Ctrl Pts',(-20.7831184061431,-18.4015323427769,
-3.14471637276859));
#76661=CARTESIAN_POINT('Ctrl Pts',(-20.7415406505033,-18.2652110975059,
-3.15226989085367));
#76662=CARTESIAN_POINT('Ctrl Pts',(-20.6575308786554,-18.0646525712234,
-3.16430917626056));
#76663=CARTESIAN_POINT('Ctrl Pts',(-20.624765051529,-17.9968238532109,-3.16856377200981));
#76664=CARTESIAN_POINT('Ctrl Pts',(-20.5838855720109,-17.9225815359599,
-3.17358685068925));
#76665=CARTESIAN_POINT('Ctrl Pts',(-20.5792539110375,-17.9143020671391,
-3.17415234859705));
#76666=CARTESIAN_POINT('Ctrl Pts',(-20.5723045530033,-17.9020731754783,
-3.17499594404416));
#76667=CARTESIAN_POINT('Ctrl Pts',(-20.5700293647512,-17.8980995600578,
-3.17527137574389));
#76668=CARTESIAN_POINT('Ctrl Pts',(-20.5659565571533,-17.8910396192182,
-3.1757631411735));
#76669=CARTESIAN_POINT('Ctrl Pts',(-20.5641640012562,-17.8879504310608,
-3.17597914657379));
#76670=CARTESIAN_POINT('Ctrl Pts',(-20.5602911281429,-17.8813148833034,
-3.17644491875611));
#76671=CARTESIAN_POINT('Ctrl Pts',(-20.5582083254959,-17.8777700951956,
-3.17669484162145));
#76672=CARTESIAN_POINT('Ctrl Pts',(-20.5524255212133,-17.8679934733214,
-3.17738713606048));
#76673=CARTESIAN_POINT('Ctrl Pts',(-20.5487038640988,-17.8617746066947,
-3.17783088201754));
#76674=CARTESIAN_POINT('Ctrl Pts',(-20.5280540698229,-17.827667617119,-3.18028270346098));
#76675=CARTESIAN_POINT('Ctrl Pts',(-20.5105159352334,-17.8001561853588,
-3.18232731782027));
#76676=CARTESIAN_POINT('Ctrl Pts',(-20.4017832506917,-17.6379845704622,
-3.19473521305806));
#76677=CARTESIAN_POINT('Ctrl Pts',(-20.2959558316742,-17.5137957579558,
-3.2056869923486));
#76678=CARTESIAN_POINT('Ctrl Pts',(-20.0915015827885,-17.32334492249,-3.22393806664416));
#76679=CARTESIAN_POINT('Ctrl Pts',(-19.9995962773085,-17.250940984881,-3.23137718247265));
#76680=CARTESIAN_POINT('Ctrl Pts',(-19.8902556552171,-17.1785947909833,
-3.23938263451834));
#76681=CARTESIAN_POINT('Ctrl Pts',(-19.8782592703425,-17.1708307453977,
-3.24025058944005));
#76682=CARTESIAN_POINT('Ctrl Pts',(-19.8590411953543,-17.1586671290977,
-3.24162487099198));
#76683=CARTESIAN_POINT('Ctrl Pts',(-19.8518703296846,-17.1541884396987,
-3.2421341255113));
#76684=CARTESIAN_POINT('Ctrl Pts',(-19.8391760166392,-17.1463653023819,
-3.24302949654675));
#76685=CARTESIAN_POINT('Ctrl Pts',(-19.8336637737645,-17.1430029643198,
-3.24341626915737));
#76686=CARTESIAN_POINT('Ctrl Pts',(-19.8222308217142,-17.1361007014649,
-3.2442143391915));
#76687=CARTESIAN_POINT('Ctrl Pts',(-19.8163080139289,-17.132564387381,-3.2446255012173));
#76688=CARTESIAN_POINT('Ctrl Pts',(-19.8010605158282,-17.1235614075287,
-3.24567822398864));
#76689=CARTESIAN_POINT('Ctrl Pts',(-19.7917109790676,-17.1181370492328,
-3.24631824335776));
#76690=CARTESIAN_POINT('Ctrl Pts',(-19.7525150540193,-17.0957960684932,
-3.24897901160294));
#76691=CARTESIAN_POINT('Ctrl Pts',(-19.7223002429932,-17.0795340385118,
-3.25097622941703));
#76692=CARTESIAN_POINT('Ctrl Pts',(-19.6425552389293,-17.0390825099004,
-3.25612059037294));
#76693=CARTESIAN_POINT('Ctrl Pts',(-19.5924513360114,-17.0160795741263,
-3.25922833882827));
#76694=CARTESIAN_POINT('Ctrl Pts',(-19.4404220489694,-16.9533469142707,
-3.26837307984706));
#76695=CARTESIAN_POINT('Ctrl Pts',(-19.336257619456,-16.9195303418129,-3.27426134412098));
#76696=CARTESIAN_POINT('Ctrl Pts',(-19.1852144053711,-16.8831327257681,
-3.28272017749787));
#76697=CARTESIAN_POINT('Ctrl Pts',(-19.1401431065128,-16.8738147887076,
-3.28523616785355));
#76698=CARTESIAN_POINT('Ctrl Pts',(-19.0730021865743,-16.8622018945177,
-3.28901511602901));
#76699=CARTESIAN_POINT('Ctrl Pts',(-19.0511416504121,-16.8587728908796,
-3.29025036235558));
#76700=CARTESIAN_POINT('Ctrl Pts',(-18.9782517117143,-16.8485075153112,
-3.29439654873523));
#76701=CARTESIAN_POINT('Ctrl Pts',(-18.9270309001987,-16.8431904595562,
-3.29735466260615));
#76702=CARTESIAN_POINT('Ctrl Pts',(-18.8670518902524,-16.8391675801266,
-3.30092257068796));
#76703=CARTESIAN_POINT('Ctrl Pts',(-18.8584285234604,-16.83864220333,-3.30143804463868));
#76704=CARTESIAN_POINT('Ctrl Pts',(-18.84534323773,-16.8379253497651,-3.3022243592258));
#76705=CARTESIAN_POINT('Ctrl Pts',(-18.8408834109855,-16.8376951783223,
-3.30249308302644));
#76706=CARTESIAN_POINT('Ctrl Pts',(-18.8328642258223,-16.8373067458879,
-3.3029776318575));
#76707=CARTESIAN_POINT('Ctrl Pts',(-18.8293051702647,-16.8371433574955,
-3.30319316669541));
#76708=CARTESIAN_POINT('Ctrl Pts',(-18.8215561750979,-16.8368072189123,
-3.30366350593958));
#76709=CARTESIAN_POINT('Ctrl Pts',(-18.8173661830889,-16.8366379355352,
-3.30391849652393));
#76710=CARTESIAN_POINT('Ctrl Pts',(-18.8055578570849,-16.8361959951855,
-3.30463895542649));
#76711=CARTESIAN_POINT('Ctrl Pts',(-18.7979386040835,-16.8359520410562,
-3.30510598370228));
#76712=CARTESIAN_POINT('Ctrl Pts',(-18.7515930262247,-16.8347186778891,
-3.30795920468723));
#76713=CARTESIAN_POINT('Ctrl Pts',(-18.7128494621799,-16.8347513305589,
-3.31039710552513));
#76714=CARTESIAN_POINT('Ctrl Pts',(-18.5834881156202,-16.8384111118236,
-3.3186659456236));
#76715=CARTESIAN_POINT('Ctrl Pts',(-18.4931085004704,-16.8467966611819,
-3.32465075205842));
#76716=CARTESIAN_POINT('Ctrl Pts',(-18.3372551817402,-16.8714261675618,
-3.33507774052121));
#76717=CARTESIAN_POINT('Ctrl Pts',(-18.2714928771618,-16.885050162914,-3.33951216991325));
#76718=CARTESIAN_POINT('Ctrl Pts',(-18.0953521885325,-16.9303703012794,
-3.35138319824012));
#76719=CARTESIAN_POINT('Ctrl Pts',(-17.9867125146762,-16.9679570315923,
-3.35868705498082));
#76720=CARTESIAN_POINT('Ctrl Pts',(-17.8685879807642,-17.019914503744,-3.36656631690883));
#76721=CARTESIAN_POINT('Ctrl Pts',(-17.8555936119012,-17.0257875089062,
-3.36743244385989));
#76722=CARTESIAN_POINT('Ctrl Pts',(-17.8349986185777,-17.0353474890338,
-3.368804387101));
#76723=CARTESIAN_POINT('Ctrl Pts',(-17.8273591816184,-17.0389493573703,
-3.36931311579913));
#76724=CARTESIAN_POINT('Ctrl Pts',(-17.8139191417624,-17.0453847044799,
-3.37020787539313));
#76725=CARTESIAN_POINT('Ctrl Pts',(-17.8081095990445,-17.0481991601912,
-3.37059455956325));
#76726=CARTESIAN_POINT('Ctrl Pts',(-17.7961156722072,-17.0540775516699,
-3.37139274724937));
#76727=CARTESIAN_POINT('Ctrl Pts',(-17.7899332089932,-17.0571452488259,
-3.37180411388749));
#76728=CARTESIAN_POINT('Ctrl Pts',(-17.7740927119444,-17.0651019701378,
-3.37285798266288));
#76729=CARTESIAN_POINT('Ctrl Pts',(-17.7644568990954,-17.0700349740666,
-3.37349893683031));
#76730=CARTESIAN_POINT('Ctrl Pts',(-17.7243188278068,-17.0909735445627,
-3.37616880653635));
#76731=CARTESIAN_POINT('Ctrl Pts',(-17.6941706645162,-17.107648978816,-3.37817398504847));
#76732=CARTESIAN_POINT('Ctrl Pts',(-17.6166171846615,-17.1530515004375,
-3.38334350621631));
#76733=CARTESIAN_POINT('Ctrl Pts',(-17.5699084499522,-17.1829178713438,
-3.38646794689538));
#76734=CARTESIAN_POINT('Ctrl Pts',(-17.434470325509,-17.2772089951712,-3.39564179683054));
#76735=CARTESIAN_POINT('Ctrl Pts',(-17.3495146403673,-17.3467263700294,
-3.40154257811789));
#76736=CARTESIAN_POINT('Ctrl Pts',(-17.2253030156092,-17.4655930736365,
-3.41090428151993));
#76737=CARTESIAN_POINT('Ctrl Pts',(-17.182208059007,-17.5106418982638,-3.41431721164908));
#76738=CARTESIAN_POINT('Ctrl Pts',(-17.1041023086802,-17.5998578597279,
-3.4209698238421));
#76739=CARTESIAN_POINT('Ctrl Pts',(-17.0687455816744,-17.6436493600893,
-3.42419174947284));
#76740=CARTESIAN_POINT('Ctrl Pts',(-17.029907751694,-17.6958803306067,-3.42805339840083));
#76741=CARTESIAN_POINT('Ctrl Pts',(-17.024681887737,-17.7030009609612,-3.42858024845712));
#76742=CARTESIAN_POINT('Ctrl Pts',(-17.0168567957713,-17.7138043238606,
-3.42938051768936));
#76743=CARTESIAN_POINT('Ctrl Pts',(-17.0142244454959,-17.7174630999822,
-3.4296517057325));
#76744=CARTESIAN_POINT('Ctrl Pts',(-17.0095306783354,-17.724031241222,-3.4301388774044));
#76745=CARTESIAN_POINT('Ctrl Pts',(-17.0074649100795,-17.7269374314379,
-3.43035455679817));
#76746=CARTESIAN_POINT('Ctrl Pts',(-17.0030039146711,-17.7332470011605,
-3.43082308993311));
#76747=CARTESIAN_POINT('Ctrl Pts',(-17.0006114106405,-17.7366521826266,
-3.43107611829161));
#76748=CARTESIAN_POINT('Ctrl Pts',(-16.9939485295931,-17.7461949631425,
-3.43178562982335));
#76749=CARTESIAN_POINT('Ctrl Pts',(-16.9897006547124,-17.752348093499,-3.43224359956881));
#76750=CARTESIAN_POINT('Ctrl Pts',(-16.9650722077977,-17.7884302411408,
-3.43493133031106));
#76751=CARTESIAN_POINT('Ctrl Pts',(-16.9454309019536,-17.8188537886966,
-3.43720621601769));
#76752=CARTESIAN_POINT('Ctrl Pts',(-16.8845074363521,-17.91875455471,-3.44466644430703));
#76753=CARTESIAN_POINT('Ctrl Pts',(-16.8464214866401,-17.9900932937538,
-3.44997665662514));
#76754=CARTESIAN_POINT('Ctrl Pts',(-16.7350512317748,-18.2309259319501,
-3.46749639804901));
#76755=CARTESIAN_POINT('Ctrl Pts',(-16.6798104289505,-18.4078709953419,
-3.47965146933822));
#76756=CARTESIAN_POINT('Ctrl Pts',(-16.6444212787081,-18.6116428570199,
-3.49237191650146));
#76757=CARTESIAN_POINT('Ctrl Pts',(-16.6409656433381,-18.633582886672,-3.49372698156557));
#76758=CARTESIAN_POINT('Ctrl Pts',(-16.6366691327942,-18.6639651841717,
-3.49558404564725));
#76759=CARTESIAN_POINT('Ctrl Pts',(-16.6355328663374,-18.6723636041767,
-3.4960953457489));
#76760=CARTESIAN_POINT('Ctrl Pts',(-16.6336677996926,-18.6868007522204,
-3.49697084922426));
#76761=CARTESIAN_POINT('Ctrl Pts',(-16.6329145422906,-18.6928361651893,
-3.49733582144025));
#76762=CARTESIAN_POINT('Ctrl Pts',(-16.6314164660555,-18.7052753673423,
-3.49808595291603));
#76763=CARTESIAN_POINT('Ctrl Pts',(-16.630674867349,-18.7116794862016,-3.49847100687257));
#76764=CARTESIAN_POINT('Ctrl Pts',(-16.6290190463627,-18.7265735221345,
-3.49936392526794));
#76765=CARTESIAN_POINT('Ctrl Pts',(-16.6281269086576,-18.7350658198487,
-3.4998710889412));
#76766=CARTESIAN_POINT('Ctrl Pts',(-16.6254426677784,-18.7621960206922,
-3.5014852204105));
#76767=CARTESIAN_POINT('Ctrl Pts',(-16.6238463997406,-18.7808527228416,
-3.50258603174766));
#76768=CARTESIAN_POINT('Ctrl Pts',(-16.6207022632528,-18.8243943390283,
-3.50513524117928));
#76769=CARTESIAN_POINT('Ctrl Pts',(-16.6193460402236,-18.8492905426304,
-3.50657769657541));
#76770=CARTESIAN_POINT('Ctrl Pts',(-16.6161241558677,-18.9369077386372,
-3.51160756551674));
#76771=CARTESIAN_POINT('Ctrl Pts',(-16.6166070346251,-18.9996842644478,
-3.51512648289882));
#76772=CARTESIAN_POINT('Ctrl Pts',(-16.6251169534667,-19.162719350435,-3.5241519935401));
#76773=CARTESIAN_POINT('Ctrl Pts',(-16.6374969846859,-19.262589640145,-3.52956469392171));
#76774=CARTESIAN_POINT('Ctrl Pts',(-16.6713133767545,-19.4342388659572,
-3.53909562781371));
#76775=CARTESIAN_POINT('Ctrl Pts',(-16.6895436984001,-19.5064613544429,
-3.54318108101848));
#76776=CARTESIAN_POINT('Ctrl Pts',(-16.7242464782779,-19.618655404559,-3.549847139363));
#76777=CARTESIAN_POINT('Ctrl Pts',(-16.7382032335146,-19.6593424542716,
-3.55233361274859));
#76778=CARTESIAN_POINT('Ctrl Pts',(-16.7560328997254,-19.7065801780384,
-3.55533297897032));
#76779=CARTESIAN_POINT('Ctrl Pts',(-16.7587148310986,-19.713573103922,-3.55577993859825));
#76780=CARTESIAN_POINT('Ctrl Pts',(-16.7631101361496,-19.724854104536,-3.55650596691035));
#76781=CARTESIAN_POINT('Ctrl Pts',(-16.7648005588927,-19.7291511323694,
-3.55678369356958));
#76782=CARTESIAN_POINT('Ctrl Pts',(-16.7678248317406,-19.736765565053,-3.55727797960094));
#76783=CARTESIAN_POINT('Ctrl Pts',(-16.7691530418488,-19.7400851573319,
-3.55749419764027));
#76784=CARTESIAN_POINT('Ctrl Pts',(-16.7720172825604,-19.7471914956494,
-3.55795864190332));
#76785=CARTESIAN_POINT('Ctrl Pts',(-16.7735558461246,-19.750977106786,-3.55820701483607));
#76786=CARTESIAN_POINT('Ctrl Pts',(-16.7778103862272,-19.7613590572156,
-3.55889076094335));
#76787=CARTESIAN_POINT('Ctrl Pts',(-16.7805487299379,-19.7679460893235,
-3.55932745424807));
#76788=CARTESIAN_POINT('Ctrl Pts',(-16.7953642529426,-19.803082467704,-3.56167177331539));
#76789=CARTESIAN_POINT('Ctrl Pts',(-16.8080334423877,-19.831376205448,-3.56361233621496));
#76790=CARTESIAN_POINT('Ctrl Pts',(-16.8914421534581,-20.0071948713133,
-3.57595985721899));
#76791=CARTESIAN_POINT('Ctrl Pts',(-16.9784616229249,-20.1463786198815,
-3.58697916217434));
#76792=CARTESIAN_POINT('Ctrl Pts',(-17.1541016996981,-20.3660178360548,
-3.60535443711196));
#76793=CARTESIAN_POINT('Ctrl Pts',(-17.2351020366533,-20.4516125960041,
-3.61284962524372));
#76794=CARTESIAN_POINT('Ctrl Pts',(-17.3334673883594,-20.5395773632765,
-3.62090722677531));
#76795=CARTESIAN_POINT('Ctrl Pts',(-17.3442230955028,-20.5490014565223,
-3.62177583862196));
#76796=CARTESIAN_POINT('Ctrl Pts',(-17.3614909775208,-20.5638249013515,
-3.62315096039115));
#76797=CARTESIAN_POINT('Ctrl Pts',(-17.3679413048689,-20.5692953268043,
-3.62366040377535));
#76798=CARTESIAN_POINT('Ctrl Pts',(-17.3793739084945,-20.5788739495618,
-3.62455599451275));
#76799=CARTESIAN_POINT('Ctrl Pts',(-17.3843424904639,-20.5829982538114,
-3.62494279897377));
#76800=CARTESIAN_POINT('Ctrl Pts',(-17.3946567976818,-20.5914805131012,
-3.6257408271769));
#76801=CARTESIAN_POINT('Ctrl Pts',(-17.400005110778,-20.595835211843,-3.62615191605153));
#76802=CARTESIAN_POINT('Ctrl Pts',(-17.4137852881771,-20.6069437519117,
-3.62720422900319));
#76803=CARTESIAN_POINT('Ctrl Pts',(-17.4222478076719,-20.6136593813945,
-3.62784391405927));
#76804=CARTESIAN_POINT('Ctrl Pts',(-17.4577578247429,-20.6413988429035,
-3.63050143480448));
#76805=CARTESIAN_POINT('Ctrl Pts',(-17.4852631032338,-20.6618300789155,
-3.63249581268312));
#76806=CARTESIAN_POINT('Ctrl Pts',(-17.5581870839315,-20.7133000397434,
-3.6376312080087));
#76807=CARTESIAN_POINT('Ctrl Pts',(-17.6043416785304,-20.7432527913602,
-3.64073301059341));
#76808=CARTESIAN_POINT('Ctrl Pts',(-17.7399452826533,-20.8239263784107,
-3.64950725668404));
#76809=CARTESIAN_POINT('Ctrl Pts',(-17.8319897860291,-20.8699759324472,
-3.65505452014676));
#76810=CARTESIAN_POINT('Ctrl Pts',(-17.9865129944676,-20.9336896684191,
-3.6641437014595));
#76811=CARTESIAN_POINT('Ctrl Pts',(-18.0470955714514,-20.9554950339264,
-3.6676573038223));
#76812=CARTESIAN_POINT('Ctrl Pts',(-18.1672384902349,-20.9926471980787,
-3.67468495367161));
#76813=CARTESIAN_POINT('Ctrl Pts',(-18.2266586984968,-21.0082254039323,
-3.67818851473783));
#76814=CARTESIAN_POINT('Ctrl Pts',(-18.2955825262409,-21.0231258648863,
-3.6823707336775));
#76815=CARTESIAN_POINT('Ctrl Pts',(-18.3045117355898,-21.0249959125553,
-3.68291480586106));
#76816=CARTESIAN_POINT('Ctrl Pts',(-18.3178694090414,-21.0277034087792,
-3.68373245776881));
#76817=CARTESIAN_POINT('Ctrl Pts',(-18.3222890479464,-21.0285845518653,
-3.68400360443394));
#76818=CARTESIAN_POINT('Ctrl Pts',(-18.3302104133595,-21.0301375515718,
-3.68449073177888));
#76819=CARTESIAN_POINT('Ctrl Pts',(-18.3337110522616,-21.030814679468,-3.68470640845911));
#76820=CARTESIAN_POINT('Ctrl Pts',(-18.3413018670186,-21.032263084386,-3.68517497062505));
#76821=CARTESIAN_POINT('Ctrl Pts',(-18.3453925563355,-21.0330311333438,
-3.68542803091718));
#76822=CARTESIAN_POINT('Ctrl Pts',(-18.3568404762853,-21.0351456107814,
-3.68613772016426));
#76823=CARTESIAN_POINT('Ctrl Pts',(-18.3642025317645,-21.0364651042164,
-3.68659583686972));
#76824=CARTESIAN_POINT('Ctrl Pts',(-18.4062226472798,-21.0437667120568,
-3.68921981782216));
#76825=CARTESIAN_POINT('Ctrl Pts',(-18.4410163913472,-21.0489230413356,
-3.69142815028951));
#76826=CARTESIAN_POINT('Ctrl Pts',(-18.5527211397596,-21.0626431204196,
-3.6985975852703));
#76827=CARTESIAN_POINT('Ctrl Pts',(-18.6299767610013,-21.0678577332487,
-3.70367415276998));
#76828=CARTESIAN_POINT('Ctrl Pts',(-18.8713067416439,-21.0708972890744,
-3.71960110373368));
#76829=CARTESIAN_POINT('Ctrl Pts',(-19.0349889865895,-21.05390413415,-3.73044991121841));
#76830=CARTESIAN_POINT('Ctrl Pts',(-19.2357062130324,-21.009112618543,-3.74331746309862));
#76831=CARTESIAN_POINT('Ctrl Pts',(-19.2760555607942,-20.9988506547641,
-3.74588521346109));
#76832=CARTESIAN_POINT('Ctrl Pts',(-19.3276857353803,-20.984085626922,-3.74914844971681));
#76833=CARTESIAN_POINT('Ctrl Pts',(-19.3392645955762,-20.9806669333192,
-3.74987882979632));
#76834=CARTESIAN_POINT('Ctrl Pts',(-19.3576800302606,-20.9750580167046,
-3.75103828548124));
#76835=CARTESIAN_POINT('Ctrl Pts',(-19.3645356759786,-20.9729317856853,
-3.75146944321166));
#76836=CARTESIAN_POINT('Ctrl Pts',(-19.3768578510903,-20.9690413421671,
-3.7522435716577));
#76837=CARTESIAN_POINT('Ctrl Pts',(-19.3823282406043,-20.9672896779768,
-3.75258694985607));
#76838=CARTESIAN_POINT('Ctrl Pts',(-19.3951462353479,-20.9631276565673,
-3.75339088208151));
#76839=CARTESIAN_POINT('Ctrl Pts',(-19.4024879291187,-20.9606992523958,
-3.75385083720906));
#76840=CARTESIAN_POINT('Ctrl Pts',(-19.4226688931911,-20.9539011192879,
-3.75511386702412));
#76841=CARTESIAN_POINT('Ctrl Pts',(-19.4354798738525,-20.9494481057738,
-3.75591418571056));
#76842=CARTESIAN_POINT('Ctrl Pts',(-19.5138716712433,-20.9213524067101,
-3.76080383739638));
#76843=CARTESIAN_POINT('Ctrl Pts',(-19.5782981884462,-20.8946041161553,
-3.76478762826629));
#76844=CARTESIAN_POINT('Ctrl Pts',(-19.7647122572798,-20.8061793341797,
-3.7763465812836));
#76845=CARTESIAN_POINT('Ctrl Pts',(-19.8821740152948,-20.7358290647983,
-3.78365452961412));
#76846=CARTESIAN_POINT('Ctrl Pts',(-20.0762780510362,-20.5924110088189,
-3.79684035205429));
#76847=CARTESIAN_POINT('Ctrl Pts',(-20.1557687662013,-20.5240134439716,
-3.80264508842154));
#76848=CARTESIAN_POINT('Ctrl Pts',(-20.2367163588933,-20.4431828791227,
-3.80942238885642));
#76849=CARTESIAN_POINT('Ctrl Pts',(-20.2435237139725,-20.4362914077689,
-3.80999964040408));
#76850=CARTESIAN_POINT('Ctrl Pts',(-20.2535060244761,-20.4260460531825,
-3.81085743565184));
#76851=CARTESIAN_POINT('Ctrl Pts',(-20.2567177954723,-20.42272799652,-3.81113518154812));
#76852=CARTESIAN_POINT('Ctrl Pts',(-20.2623970491556,-20.4168222570494,
-3.81162948880734));
#76853=CARTESIAN_POINT('Ctrl Pts',(-20.2648688595173,-20.4142388038092,
-3.81184570872853));
#76854=CARTESIAN_POINT('Ctrl Pts',(-20.2701515051174,-20.4086894830196,
-3.81231014231393));
#76855=CARTESIAN_POINT('Ctrl Pts',(-20.2729602595526,-20.4057217806305,
-3.81255850261044));
#76856=CARTESIAN_POINT('Ctrl Pts',(-20.2787067622919,-20.3996147637823,
-3.81306952369131));
#76857=CARTESIAN_POINT('Ctrl Pts',(-20.2816435723938,-20.3964745957892,
-3.81333225270047));
#76858=CARTESIAN_POINT('Ctrl Pts',(-20.2951037388432,-20.3819942163683,
-3.81454354142486));
#76859=CARTESIAN_POINT('Ctrl Pts',(-20.3055118358505,-20.3705481521945,
-3.81550032218878));
#76860=CARTESIAN_POINT('Ctrl Pts',(-20.3738183655828,-20.2937552486411,
-3.82190882332335));
#76861=CARTESIAN_POINT('Ctrl Pts',(-20.4277468291377,-20.2250003784039,
-3.82759284987748));
#76862=CARTESIAN_POINT('Ctrl Pts',(-20.5185513242836,-20.0932094601856,
-3.83812777718336));
#76863=CARTESIAN_POINT('Ctrl Pts',(-20.5567150918504,-20.0312091104248,
-3.84295349355964));
#76864=CARTESIAN_POINT('Ctrl Pts',(-20.5939227256405,-19.9631378145699,
-3.84805527367092));
#76865=CARTESIAN_POINT('Ctrl Pts',(-20.596219730547,-19.9589011375566,-3.84837202744986));
#76866=CARTESIAN_POINT('Ctrl Pts',(-20.6464310200096,-19.8655301285701,
-3.85533558745032));
#76867=CARTESIAN_POINT('Ctrl Pts',(-20.6878922366713,-19.7731104590378,
-3.86187259304192));
#76868=CARTESIAN_POINT('Ctrl Pts',(-20.7225805144725,-19.6781105545716,
-3.86819367631211));
#76869=CARTESIAN_POINT('',(-20.8509991606888,-18.9501148891277,-2.8890562790225));
#76870=CARTESIAN_POINT('Ctrl Pts',(-20.7225805821191,-19.6781103693095,
-3.64442446878243));
#76871=CARTESIAN_POINT('Ctrl Pts',(-20.6975861564812,-19.7465619871152,
-3.64005128426942));
#76872=CARTESIAN_POINT('Ctrl Pts',(-20.6690382082784,-19.8137627604839,
-3.63567809975641));
#76873=CARTESIAN_POINT('Ctrl Pts',(-20.6370917484072,-19.8793245371199,
-3.63130491524341));
#76874=CARTESIAN_POINT('Ctrl Pts',(-20.6051516095213,-19.944873341582,-3.62693259601674));
#76875=CARTESIAN_POINT('Ctrl Pts',(-20.5698145058605,-20.0087833599342,
-3.62256027679008));
#76876=CARTESIAN_POINT('Ctrl Pts',(-20.5312826026733,-20.070688627871,-3.61818795756341));
#76877=CARTESIAN_POINT('Ctrl Pts',(-20.4927456129338,-20.1326020678512,
-3.6138150611519));
#76878=CARTESIAN_POINT('Ctrl Pts',(-20.4510132433513,-20.1925098238232,
-3.6094421647404));
#76879=CARTESIAN_POINT('Ctrl Pts',(-20.4063315108142,-20.2500740802966,
-3.60506926832889));
#76880=CARTESIAN_POINT('Ctrl Pts',(-20.3616004942757,-20.3077018302098,
-3.6006915486077));
#76881=CARTESIAN_POINT('Ctrl Pts',(-20.3139139201605,-20.3629805414553,
-3.59631382888651));
#76882=CARTESIAN_POINT('Ctrl Pts',(-20.2635581471404,-20.4156054367611,
-3.59193610916532));
#76883=CARTESIAN_POINT('Ctrl Pts',(-20.2131700667217,-20.4682640952952,
-3.5875555807744));
#76884=CARTESIAN_POINT('Ctrl Pts',(-20.16010973072,-20.5182652193778,-3.58317505238349));
#76885=CARTESIAN_POINT('Ctrl Pts',(-20.1046984520788,-20.5653427265987,
-3.57879452399257));
#76886=CARTESIAN_POINT('Ctrl Pts',(-20.0491943887079,-20.612499063868,-3.57440666052201));
#76887=CARTESIAN_POINT('Ctrl Pts',(-19.9913319107465,-20.6567217240253,
-3.57001879705145));
#76888=CARTESIAN_POINT('Ctrl Pts',(-19.931462615983,-20.6977870097246,-3.56563093358088));
#76889=CARTESIAN_POINT('Ctrl Pts',(-19.9100485962753,-20.7124752207807,
-3.56406148474731));
#76890=CARTESIAN_POINT('Ctrl Pts',(-19.8883780714084,-20.7267599186563,
-3.56249203591374));
#76891=CARTESIAN_POINT('Ctrl Pts',(-19.8664678605235,-20.7406323112595,
-3.56092258708016));
#76892=CARTESIAN_POINT('Ctrl Pts',(-19.8052064921928,-20.7794197860744,
-3.55653437814988));
#76893=CARTESIAN_POINT('Ctrl Pts',(-19.7418305075798,-20.8151319931224,
-3.55214616921959));
#76894=CARTESIAN_POINT('Ctrl Pts',(-19.6766813842659,-20.8475318007774,
-3.54775796028931));
#76895=CARTESIAN_POINT('Ctrl Pts',(-19.611628953053,-20.8798835217459,-3.54337626418866));
#76896=CARTESIAN_POINT('Ctrl Pts',(-19.5448090356316,-20.908932389527,-3.53899456808801));
#76897=CARTESIAN_POINT('Ctrl Pts',(-19.4765908557835,-20.93448526373,-3.53461287198737));
#76898=CARTESIAN_POINT('Ctrl Pts',(-19.4084528377259,-20.9600081112722,
-3.53023632472836));
#76899=CARTESIAN_POINT('Ctrl Pts',(-19.3389202706952,-20.982042957579,-3.52585977746935));
#76900=CARTESIAN_POINT('Ctrl Pts',(-19.2683841301347,-21.0004439463798,
-3.52148323021034));
#76901=CARTESIAN_POINT('Ctrl Pts',(-19.1978927225695,-21.018833265541,-3.517109458494));
#76902=CARTESIAN_POINT('Ctrl Pts',(-19.1263994698856,-21.033593178237,-3.51273568677766));
#76903=CARTESIAN_POINT('Ctrl Pts',(-19.054311001005,-21.0446275021215,-3.50836191506133));
#76904=CARTESIAN_POINT('Ctrl Pts',(-18.9822444688877,-21.0556584682242,
-3.50398947429841));
#76905=CARTESIAN_POINT('Ctrl Pts',(-18.9095835567029,-21.0629660233357,
-3.4996170335355));
#76906=CARTESIAN_POINT('Ctrl Pts',(-18.8367439345943,-21.0665053047709,
-3.49524459277259));
#76907=CARTESIAN_POINT('Ctrl Pts',(-18.7639024499686,-21.0700446767059,
-3.49087204020588));
#76908=CARTESIAN_POINT('Ctrl Pts',(-18.6908827282527,-21.0698155622467,
-3.48649948763918));
#76909=CARTESIAN_POINT('Ctrl Pts',(-18.6181027067733,-21.0658251624538,
-3.48212693507248));
#76910=CARTESIAN_POINT('Ctrl Pts',(-18.5452471514426,-21.0618306212735,
-3.47774984450579));
#76911=CARTESIAN_POINT('Ctrl Pts',(-18.4726322757191,-21.0540670274163,
-3.47337275393911));
#76912=CARTESIAN_POINT('Ctrl Pts',(-18.4006723159509,-21.0425936130789,
-3.46899566337243));
#76913=CARTESIAN_POINT('Ctrl Pts',(-18.3286730561778,-21.0311139326842,
-3.46461618231413));
#76914=CARTESIAN_POINT('Ctrl Pts',(-18.2573298966098,-21.0159204984676,
-3.46023670125583));
#76915=CARTESIAN_POINT('Ctrl Pts',(-18.1870456019981,-20.997123440408,-3.45585722019753));
#76916=CARTESIAN_POINT('Ctrl Pts',(-18.1166367289457,-20.9782930646892,
-3.45146997653845));
#76917=CARTESIAN_POINT('Ctrl Pts',(-18.0472909281431,-20.9558464584345,
-3.44708273287937));
#76918=CARTESIAN_POINT('Ctrl Pts',(-17.9793940004957,-20.9299430693304,
-3.44269548922029));
#76919=CARTESIAN_POINT('Ctrl Pts',(-17.9332306321329,-20.912331260748,-3.43971258627977));
#76920=CARTESIAN_POINT('Ctrl Pts',(-17.8877366290251,-20.8931225055476,
-3.43672968333925));
#76921=CARTESIAN_POINT('Ctrl Pts',(-17.8430266573744,-20.8723789997629,
-3.43374678039873));
#76922=CARTESIAN_POINT('Ctrl Pts',(-17.7772529124841,-20.841862808246,-3.42935857146461));
#76923=CARTESIAN_POINT('Ctrl Pts',(-17.7129203794316,-20.8079039749603,
-3.42497036253048));
#76924=CARTESIAN_POINT('Ctrl Pts',(-17.6504132837259,-20.770661273661,-3.42058215359636));
#76925=CARTESIAN_POINT('Ctrl Pts',(-17.5879989589138,-20.7334738467052,
-3.41620045749186));
#76926=CARTESIAN_POINT('Ctrl Pts',(-17.5274051041874,-20.6930124717674,
-3.41181876138736));
#76927=CARTESIAN_POINT('Ctrl Pts',(-17.4689939738807,-20.6494830643873,
-3.40743706528285));
#76928=CARTESIAN_POINT('Ctrl Pts',(-17.4106514813006,-20.6060048075252,
-3.40306051801998));
#76929=CARTESIAN_POINT('Ctrl Pts',(-17.3544870028669,-20.5594659667512,
-3.39868397075711));
#76930=CARTESIAN_POINT('Ctrl Pts',(-17.300834808213,-20.5101163413077,-3.39430742349424));
#76931=CARTESIAN_POINT('Ctrl Pts',(-17.2472166390012,-20.4607980126794,
-3.38993365177404));
#76932=CARTESIAN_POINT('Ctrl Pts',(-17.1961079465045,-20.4086727619658,
-3.38555988005384));
#76933=CARTESIAN_POINT('Ctrl Pts',(-17.1478097053784,-20.3540304380606,
-3.38118610833364));
#76934=CARTESIAN_POINT('Ctrl Pts',(-17.0995261615695,-20.2994047419982,
-3.37681366756687));
#76935=CARTESIAN_POINT('Ctrl Pts',(-17.0540516905098,-20.2422638546093,
-3.3724412268001));
#76936=CARTESIAN_POINT('Ctrl Pts',(-17.011649008983,-20.1829330053837,-3.36806878603333));
#76937=CARTESIAN_POINT('Ctrl Pts',(-16.9692452432152,-20.1236006390618,
-3.36369623346278));
#76938=CARTESIAN_POINT('Ctrl Pts',(-16.9299137017783,-20.0620785933411,
-3.35932368089223));
#76939=CARTESIAN_POINT('Ctrl Pts',(-16.8938745512684,-19.9987221851716,
-3.35495112832168));
#76940=CARTESIAN_POINT('Ctrl Pts',(-16.8577979979692,-19.9353000233327,
-3.35057403775118));
#76941=CARTESIAN_POINT('Ctrl Pts',(-16.8250208968183,-19.870040118225,-3.34619694718069));
#76942=CARTESIAN_POINT('Ctrl Pts',(-16.7957176611905,-19.8033228383283,
-3.3418198566102));
#76943=CARTESIAN_POINT('Ctrl Pts',(-16.7663984219784,-19.7365691216491,
-3.33744037554812));
#76944=CARTESIAN_POINT('Ctrl Pts',(-16.7405569966193,-19.6683568969041,
-3.33306089448603));
#76945=CARTESIAN_POINT('Ctrl Pts',(-16.7183187921505,-19.5990844367796,
-3.32868141342394));
#76946=CARTESIAN_POINT('Ctrl Pts',(-16.696041170614,-19.5296891916857,-3.32429416976114));
#76947=CARTESIAN_POINT('Ctrl Pts',(-16.6773796475294,-19.4592304251164,
-3.31990692609834));
#76948=CARTESIAN_POINT('Ctrl Pts',(-16.6624089793388,-19.3881188405882,
-3.31551968243554));
#76949=CARTESIAN_POINT('Ctrl Pts',(-16.6522303676446,-19.3397698159047,
-3.31253677952946));
#76950=CARTESIAN_POINT('Ctrl Pts',(-16.6437568500116,-19.2911192245629,
-3.30955387662337));
#76951=CARTESIAN_POINT('Ctrl Pts',(-16.6369981960583,-19.2422971482212,
-3.30657097371729));
#76952=CARTESIAN_POINT('Ctrl Pts',(-16.6270554032346,-19.1704740021266,
-3.30218276479085));
#76953=CARTESIAN_POINT('Ctrl Pts',(-16.6207874279489,-19.0979992504155,
-3.29779455586441));
#76954=CARTESIAN_POINT('Ctrl Pts',(-16.6182687405808,-19.0252819071572,
-3.29340634693797));
#76955=CARTESIAN_POINT('Ctrl Pts',(-16.6157537913624,-18.9526724884929,
-3.28902465084115));
#76956=CARTESIAN_POINT('Ctrl Pts',(-16.6169771002007,-18.8798216711257,
-3.28464295474433));
#76957=CARTESIAN_POINT('Ctrl Pts',(-16.6219616061142,-18.8071455117975,
-3.2802612586475));
#76958=CARTESIAN_POINT('Ctrl Pts',(-16.6269402548367,-18.7345547527397,
-3.27588471139227));
#76959=CARTESIAN_POINT('Ctrl Pts',(-16.6356712880177,-18.6621387228747,
-3.27150816413703));
#76960=CARTESIAN_POINT('Ctrl Pts',(-16.6481255978391,-18.590313701656,-3.2671316168818));
#76961=CARTESIAN_POINT('Ctrl Pts',(-16.6605720093183,-18.5185342308214,
-3.2627578451692));
#76962=CARTESIAN_POINT('Ctrl Pts',(-16.6767369302051,-18.4473454990794,
-3.2583840734566));
#76963=CARTESIAN_POINT('Ctrl Pts',(-16.6965395553225,-18.3771574681928,
-3.254010301744));
#76964=CARTESIAN_POINT('Ctrl Pts',(-16.7163361544347,-18.3069907957591,
-3.24963786098479));
#76965=CARTESIAN_POINT('Ctrl Pts',(-16.7397681292052,-18.2378246835963,
-3.24526542022559));
#76966=CARTESIAN_POINT('Ctrl Pts',(-16.7667042167146,-18.1700560754968,
-3.24089297946638));
#76967=CARTESIAN_POINT('Ctrl Pts',(-16.793640992983,-18.1022857345459,-3.23652042690334));
#76968=CARTESIAN_POINT('Ctrl Pts',(-16.8240818798525,-18.0359134161329,
-3.23214787434029));
#76969=CARTESIAN_POINT('Ctrl Pts',(-16.8578472840016,-17.971316571848,-3.22777532177725));
#76970=CARTESIAN_POINT('Ctrl Pts',(-16.8916477311615,-17.9066526865202,
-3.22339823121414));
#76971=CARTESIAN_POINT('Ctrl Pts',(-16.9287793604406,-17.8437683827164,
-3.21902114065103));
#76972=CARTESIAN_POINT('Ctrl Pts',(-16.9690167487947,-17.7830162007262,
-3.21464405008791));
#76973=CARTESIAN_POINT('Ctrl Pts',(-17.0092761122804,-17.7222308397138,
-3.21026456903314));
#76974=CARTESIAN_POINT('Ctrl Pts',(-17.0526443249034,-17.6635803070146,
-3.20588508797837));
#76975=CARTESIAN_POINT('Ctrl Pts',(-17.0988543828141,-17.6073856275506,
-3.2015056069236));
#76976=CARTESIAN_POINT('Ctrl Pts',(-17.1451463477434,-17.5510913433929,
-3.19711836326793));
#76977=CARTESIAN_POINT('Ctrl Pts',(-17.194289891427,-17.4972619617608,-3.19273111961227));
#76978=CARTESIAN_POINT('Ctrl Pts',(-17.2459801414474,-17.4461826470143,
-3.1883438759566));
#76979=CARTESIAN_POINT('Ctrl Pts',(-17.2811245310897,-17.4114536344943,
-3.18536097298302));
#76980=CARTESIAN_POINT('Ctrl Pts',(-17.3174454256972,-17.3779951039873,
-3.18237807000944));
#76981=CARTESIAN_POINT('Ctrl Pts',(-17.3548387352824,-17.345885680936,-3.17939516703586));
#76982=CARTESIAN_POINT('Ctrl Pts',(-17.4098487897263,-17.2986488589,-3.17500695810765));
#76983=CARTESIAN_POINT('Ctrl Pts',(-17.4673958504111,-17.2541492751002,
-3.17061874917943));
#76984=CARTESIAN_POINT('Ctrl Pts',(-17.5271763106365,-17.2126709388989,
-3.16623054025122));
#76985=CARTESIAN_POINT('Ctrl Pts',(-17.5868680467463,-17.1712541634263,
-3.16184884415269));
#76986=CARTESIAN_POINT('Ctrl Pts',(-17.6487862091489,-17.1328500068486,
-3.15746714805417));
#76987=CARTESIAN_POINT('Ctrl Pts',(-17.7125933764223,-17.0977029608739,
-3.15308545195564));
#76988=CARTESIAN_POINT('Ctrl Pts',(-17.7763255651952,-17.062597215476,-3.14870890469881));
#76989=CARTESIAN_POINT('Ctrl Pts',(-17.8419419289074,-17.0307412091789,
-3.14433235744198));
#76990=CARTESIAN_POINT('Ctrl Pts',(-17.9090766869066,-17.0023357910874,
-3.13995581018516));
#76991=CARTESIAN_POINT('Ctrl Pts',(-17.9761688690172,-16.9739483872994,
-3.13558203847104));
#76992=CARTESIAN_POINT('Ctrl Pts',(-18.044777091654,-16.9490074173241,-3.13120826675692));
#76993=CARTESIAN_POINT('Ctrl Pts',(-18.1145129035424,-16.9276668413222,
-3.1268344950428));
#76994=CARTESIAN_POINT('Ctrl Pts',(-18.1842274945885,-16.9063327593294,
-3.12246205428213));
#76995=CARTESIAN_POINT('Ctrl Pts',(-18.2550685326835,-16.8885970372536,
-3.11808961352147));
#76996=CARTESIAN_POINT('Ctrl Pts',(-18.3266312007869,-16.8745641618987,
-3.11371717276081));
#76997=CARTESIAN_POINT('Ctrl Pts',(-18.3981956987552,-16.8605309277218,
-3.10934462019639));
#76998=CARTESIAN_POINT('Ctrl Pts',(-18.4704813896195,-16.8502008191088,
-3.10497206763197));
#76999=CARTESIAN_POINT('Ctrl Pts',(-18.543073685867,-16.8436271338846,-3.10059951506755));
#77000=CARTESIAN_POINT('Ctrl Pts',(-18.6157413211371,-16.837046626242,-3.09622242450318));
#77001=CARTESIAN_POINT('Ctrl Pts',(-18.6887157156715,-16.8342303693191,
-3.09184533393881));
#77002=CARTESIAN_POINT('Ctrl Pts',(-18.7615784216589,-16.8351796413822,
-3.08746824337444));
#77003=CARTESIAN_POINT('Ctrl Pts',(-18.8344809206741,-16.8361294318779,
-3.08308876231848));
#77004=CARTESIAN_POINT('Ctrl Pts',(-18.9072711279966,-16.8408488145899,
-3.07870928126251));
#77005=CARTESIAN_POINT('Ctrl Pts',(-18.9795345883502,-16.8492870462368,
-3.07432980020655));
#77006=CARTESIAN_POINT('Ctrl Pts',(-19.0519261352023,-16.8577402345926,
-3.06994255654981));
#77007=CARTESIAN_POINT('Ctrl Pts',(-19.1237885946052,-16.8699253543973,
-3.06555531289307));
#77008=CARTESIAN_POINT('Ctrl Pts',(-19.194717166803,-16.885740410255,-3.06116806923633));
#77009=CARTESIAN_POINT('Ctrl Pts',(-19.2429417616867,-16.8964931244035,
-3.05818516627569));
#77010=CARTESIAN_POINT('Ctrl Pts',(-19.2907349020831,-16.9089227808444,
-3.05520226331506));
#77011=CARTESIAN_POINT('Ctrl Pts',(-19.3379741345032,-16.9229844148329,
-3.05221936035442));
#77012=CARTESIAN_POINT('Ctrl Pts',(-19.4074687259721,-16.9436707693596,
-3.04783115140139));
#77013=CARTESIAN_POINT('Ctrl Pts',(-19.4760349665996,-16.9679719598249,
-3.04344294244835));
#77014=CARTESIAN_POINT('Ctrl Pts',(-19.5432697129059,-16.995786429918,-3.03905473349532));
#77015=CARTESIAN_POINT('Ctrl Pts',(-19.6104046717026,-17.0235596187263,
-3.03467303737184));
#77016=CARTESIAN_POINT('Ctrl Pts',(-19.6762116170654,-17.054835553211,-3.03029134124837));
#77017=CARTESIAN_POINT('Ctrl Pts',(-19.7403023303408,-17.0894628540749,
-3.02590964512489));
#77018=CARTESIAN_POINT('Ctrl Pts',(-19.8043177319278,-17.1240494651048,
-3.02153309784305));
#77019=CARTESIAN_POINT('Ctrl Pts',(-19.8666204853438,-17.1619793912516,
-3.0171565505612));
#77020=CARTESIAN_POINT('Ctrl Pts',(-19.9268437181447,-17.2030537846799,
-3.01278000327936));
#77021=CARTESIAN_POINT('Ctrl Pts',(-19.9870287582467,-17.2441021293248,
-3.00840623154019));
#77022=CARTESIAN_POINT('Ctrl Pts',(-20.0451364968745,-17.2882907134169,
-3.00403245980103));
#77023=CARTESIAN_POINT('Ctrl Pts',(-20.100827216588,-17.3353762466194,-2.99965868806186));
#77024=CARTESIAN_POINT('Ctrl Pts',(-20.156500989428,-17.3824474515356,-2.99528624727616));
#77025=CARTESIAN_POINT('Ctrl Pts',(-20.2097588354208,-17.4324135441543,
-2.99091380649046));
#77026=CARTESIAN_POINT('Ctrl Pts',(-20.2602937779114,-17.48499069413,-2.98654136570476));
#77027=CARTESIAN_POINT('Ctrl Pts',(-20.3108300125851,-17.5375691885083,
-2.98216881311535));
#77028=CARTESIAN_POINT('Ctrl Pts',(-20.3586428726932,-17.5927585236335,
-2.97779626052593));
#77029=CARTESIAN_POINT('Ctrl Pts',(-20.40346313484,-17.6502389461156,-2.97342370793652));
#77030=CARTESIAN_POINT('Ctrl Pts',(-20.4483299131425,-17.7077790239444,
-2.96904661734739));
#77031=CARTESIAN_POINT('Ctrl Pts',(-20.4901975952304,-17.7676145553053,
-2.96466952675826));
#77032=CARTESIAN_POINT('Ctrl Pts',(-20.5288386084183,-17.8293943837077,
-2.96029243616913));
#77033=CARTESIAN_POINT('Ctrl Pts',(-20.5675007248966,-17.8912079523656,
-2.9559129550885));
#77034=CARTESIAN_POINT('Ctrl Pts',(-20.6029324294701,-17.9549675102643,
-2.95153347400787));
#77035=CARTESIAN_POINT('Ctrl Pts',(-20.6349520524258,-18.0202970997264,
-2.94715399292724));
#77036=CARTESIAN_POINT('Ctrl Pts',(-20.6670284299448,-18.0857424854403,
-2.94276674924626));
#77037=CARTESIAN_POINT('Ctrl Pts',(-20.695680458665,-18.1527630160604,-2.93837950556528));
#77038=CARTESIAN_POINT('Ctrl Pts',(-20.7207747901411,-18.2209631108763,
-2.9339922618843));
#77039=CARTESIAN_POINT('Ctrl Pts',(-20.7378365162473,-18.2673326003074,
-2.9310093591472));
#77040=CARTESIAN_POINT('Ctrl Pts',(-20.7532546613818,-18.3142470017661,
-2.92802645641009));
#77041=CARTESIAN_POINT('Ctrl Pts',(-20.767000752034,-18.3615790127128,-2.92504355367299));
#77042=CARTESIAN_POINT('Ctrl Pts',(-20.7921933233422,-18.4483247712785,
-2.91957676374621));
#77043=CARTESIAN_POINT('Ctrl Pts',(-20.8118478930265,-18.5367464915126,
-2.91410997381944));
#77044=CARTESIAN_POINT('Ctrl Pts',(-20.8257819138148,-18.6262126076147,
-2.90864318389266));
#77045=CARTESIAN_POINT('Ctrl Pts',(-20.8394880731057,-18.7142156942372,
-2.90326579177559));
#77046=CARTESIAN_POINT('Ctrl Pts',(-20.8476592207529,-18.8032293912446,
-2.89788839965851));
#77047=CARTESIAN_POINT('Ctrl Pts',(-20.8501673751625,-18.8926313188794,
-2.89251100754144));
#77048=CARTESIAN_POINT('Ctrl Pts',(-20.8507044999979,-18.911776868886,-2.89135943136846));
#77049=CARTESIAN_POINT('Ctrl Pts',(-20.8509820862726,-18.9309401417771,
-2.89020785519548));
#77050=CARTESIAN_POINT('Ctrl Pts',(-20.8509991606888,-18.9501148891277,
-2.8890562790225));
#77051=CARTESIAN_POINT('Ctrl Pts',(-20.849962012661,-18.9501158126703,-2.8890562790225));
#77052=CARTESIAN_POINT('Ctrl Pts',(-20.8478498624177,-19.1969462894927,
-2.87422526082294));
#77053=CARTESIAN_POINT('Ctrl Pts',(-20.8034779929369,-19.4444419793215,
-2.85939424262338));
#77054=CARTESIAN_POINT('Ctrl Pts',(-20.7202230519095,-19.6772708889146,
-2.84456322442383));
#77055=CARTESIAN_POINT('Origin',(-18.734,-18.952,0.));
#77056=CARTESIAN_POINT('',(-20.7225805826894,-19.6781103677477,-2.04625070052543));
#77057=CARTESIAN_POINT('',(-20.7225805820961,-19.6781103693727,-2.26547392846891));
#77058=CARTESIAN_POINT('',(-20.7225805821191,-19.6781103693095,0.));
#77059=CARTESIAN_POINT('',(-20.8509992561133,-18.9537747157296,-2.31031853654595));
#77060=CARTESIAN_POINT('Ctrl Pts',(-20.7225805820961,-19.6781103693727,
-2.26547392846891));
#77061=CARTESIAN_POINT('Ctrl Pts',(-20.7575267620676,-19.5824041271247,
-2.2710458239064));
#77062=CARTESIAN_POINT('Ctrl Pts',(-20.7855141340195,-19.4843107263304,
-2.27670326525148));
#77063=CARTESIAN_POINT('Ctrl Pts',(-20.8083091787163,-19.3751126538042,
-2.2833121262572));
#77064=CARTESIAN_POINT('Ctrl Pts',(-20.8102239943213,-19.3656143180092,
-2.28388953700015));
#77065=CARTESIAN_POINT('Ctrl Pts',(-20.8129550917444,-19.3515698395547,
-2.2847475243896));
#77066=CARTESIAN_POINT('Ctrl Pts',(-20.8138218385678,-19.3470334784062,
-2.28502530142322));
#77067=CARTESIAN_POINT('Ctrl Pts',(-20.8153332698376,-19.3389801091439,
-2.28551964303392));
#77068=CARTESIAN_POINT('Ctrl Pts',(-20.8159838956222,-19.3354642658266,
-2.2857358659928));
#77069=CARTESIAN_POINT('Ctrl Pts',(-20.8173589190641,-19.3279272645982,
-2.2862002822975));
#77070=CARTESIAN_POINT('Ctrl Pts',(-20.8180805726934,-19.3239057135641,
-2.28644862215127));
#77071=CARTESIAN_POINT('Ctrl Pts',(-20.819537639316,-19.3156485071271,-2.28695959356709));
#77072=CARTESIAN_POINT('Ctrl Pts',(-20.8202718006576,-19.3114126525071,
-2.28722229330262));
#77073=CARTESIAN_POINT('Ctrl Pts',(-20.8220971202441,-19.3006871419385,
-2.28788887808368));
#77074=CARTESIAN_POINT('Ctrl Pts',(-20.823170921096,-19.2941946323735,-2.28829368782551));
#77075=CARTESIAN_POINT('Ctrl Pts',(-20.8419517333718,-19.1772561807361,
-2.29560698829358));
#77076=CARTESIAN_POINT('Ctrl Pts',(-20.8509055123085,-19.0655985766051,
-2.30293678580813));
#77077=CARTESIAN_POINT('Ctrl Pts',(-20.8509992561133,-18.9537747157296,
-2.31031853654595));
#77078=CARTESIAN_POINT('Ctrl Pts',(-20.8509992546724,-18.9537764337049,
-2.31031842313845));
#77079=CARTESIAN_POINT('Ctrl Pts',(-20.8510843034766,-18.8524226625882,
-2.31700901865283));
#77080=CARTESIAN_POINT('Ctrl Pts',(-20.8438905426111,-18.7511845230255,
-2.32372474899395));
#77081=CARTESIAN_POINT('Ctrl Pts',(-20.8169301667289,-18.563591183208,-2.33599520132961));
#77082=CARTESIAN_POINT('Ctrl Pts',(-20.7989516822577,-18.4771974729164,
-2.34157662375898));
#77083=CARTESIAN_POINT('Ctrl Pts',(-20.7702116745163,-18.3723866086643,
-2.34824632884448));
#77084=CARTESIAN_POINT('Ctrl Pts',(-20.7645005235169,-18.3526859443344,
-2.34949575392107));
#77085=CARTESIAN_POINT('Ctrl Pts',(-20.75591384801,-18.3245991161562,-2.35127147777804));
#77086=CARTESIAN_POINT('Ctrl Pts',(-20.7532707044411,-18.3161436453596,
-2.35180533073409));
#77087=CARTESIAN_POINT('Ctrl Pts',(-20.7485964764223,-18.3015138128981,
-2.3527278285672));
#77088=CARTESIAN_POINT('Ctrl Pts',(-20.7465899039902,-18.2953318020169,
-2.3531172723558));
#77089=CARTESIAN_POINT('Ctrl Pts',(-20.7426769449974,-18.2834628625813,
-2.35386429785767));
#77090=CARTESIAN_POINT('Ctrl Pts',(-20.7407748004187,-18.2777746111156,
-2.35422201494289));
#77091=CARTESIAN_POINT('Ctrl Pts',(-20.7357282855469,-18.2628938705469,
-2.35515707901907));
#77092=CARTESIAN_POINT('Ctrl Pts',(-20.7325447424454,-18.2537147402154,
-2.3557331260957));
#77093=CARTESIAN_POINT('Ctrl Pts',(-20.7212756715466,-18.2219310080391,
-2.35772543262704));
#77094=CARTESIAN_POINT('Ctrl Pts',(-20.712868733493,-18.1994417414467,-2.35913101792212));
#77095=CARTESIAN_POINT('Ctrl Pts',(-20.6489791070301,-18.0370108868283,
-2.36926326534927));
#77096=CARTESIAN_POINT('Ctrl Pts',(-20.579092299269,-17.9031953293941,-2.37746165698123));
#77097=CARTESIAN_POINT('Ctrl Pts',(-20.4589031767015,-17.7228643216449,
-2.38923025126843));
#77098=CARTESIAN_POINT('Ctrl Pts',(-20.419654497017,-17.6695671941733,-2.39281850192715));
#77099=CARTESIAN_POINT('Ctrl Pts',(-20.3433815131489,-17.5755570867321,
-2.39950740498086));
#77100=CARTESIAN_POINT('Ctrl Pts',(-20.3071431999893,-17.5342822619525,
-2.40258503118372));
#77101=CARTESIAN_POINT('Ctrl Pts',(-20.2498839317676,-17.4739662245475,
-2.40738294988533));
#77102=CARTESIAN_POINT('Ctrl Pts',(-20.2300158975193,-17.4538597547527,
-2.40903691680933));
#77103=CARTESIAN_POINT('Ctrl Pts',(-20.204871379837,-17.4294124884789,-2.41112625537063));
#77104=CARTESIAN_POINT('Ctrl Pts',(-20.1999675447591,-17.4246904370405,
-2.41153355304756));
#77105=CARTESIAN_POINT('Ctrl Pts',(-20.1920749587726,-17.4171634568076,
-2.41218897213734));
#77106=CARTESIAN_POINT('Ctrl Pts',(-20.189100642402,-17.4143433674762,-2.41243594049324));
#77107=CARTESIAN_POINT('Ctrl Pts',(-20.183517820333,-17.4090807347955,-2.41289949705779));
#77108=CARTESIAN_POINT('Ctrl Pts',(-20.1809113134251,-17.4066361526108,
-2.41311592397766));
#77109=CARTESIAN_POINT('Ctrl Pts',(-20.1749367418387,-17.4010611070537,
-2.41361200686093));
#77110=CARTESIAN_POINT('Ctrl Pts',(-20.1715646701594,-17.3979350200772,
-2.41389199041614));
#77111=CARTESIAN_POINT('Ctrl Pts',(-20.1611317026697,-17.3883261251821,
-2.4147581416011));
#77112=CARTESIAN_POINT('Ctrl Pts',(-20.1540370547588,-17.3818803743891,
-2.41534700356176));
#77113=CARTESIAN_POINT('Ctrl Pts',(-20.0609538422547,-17.2984577440783,
-2.42306828895633));
#77114=CARTESIAN_POINT('Ctrl Pts',(-19.9688635983804,-17.2285980909303,
-2.43064533735236));
#77115=CARTESIAN_POINT('Ctrl Pts',(-19.7568270044209,-17.093500790107,-2.44724911310532));
#77116=CARTESIAN_POINT('Ctrl Pts',(-19.6353076822509,-17.0316232020963,
-2.45624208495786));
#77117=CARTESIAN_POINT('Ctrl Pts',(-19.4515627171354,-16.9593736994179,
-2.46876543184455));
#77118=CARTESIAN_POINT('Ctrl Pts',(-19.3934914252173,-16.9394076171203,
-2.47258367441128));
#77119=CARTESIAN_POINT('Ctrl Pts',(-19.3220865375304,-16.9182806677852,
-2.47711488452111));
#77120=CARTESIAN_POINT('Ctrl Pts',(-19.3095092614356,-16.9146857876376,
-2.47790702471601));
#77121=CARTESIAN_POINT('Ctrl Pts',(-19.2897662094287,-16.9092401825917,
-2.47914131244906));
#77122=CARTESIAN_POINT('Ctrl Pts',(-19.2826228345554,-16.907310111843,-2.47958603105056));
#77123=CARTESIAN_POINT('Ctrl Pts',(-19.2699384595304,-16.9039541752115,
-2.48037244931891));
#77124=CARTESIAN_POINT('Ctrl Pts',(-19.2644015525042,-16.9025132528038,
-2.48071463394917));
#77125=CARTESIAN_POINT('Ctrl Pts',(-19.2516307390168,-16.8992450012206,
-2.48150138269828));
#77126=CARTESIAN_POINT('Ctrl Pts',(-19.2443928501979,-16.8974334258437,
-2.48194543380327));
#77127=CARTESIAN_POINT('Ctrl Pts',(-19.2245130458354,-16.8925692331332,
-2.4831601256031));
#77128=CARTESIAN_POINT('Ctrl Pts',(-19.2118522090242,-16.889594751431,-2.48392824569442));
#77129=CARTESIAN_POINT('Ctrl Pts',(-19.1470884397097,-16.8750078389006,
-2.48783049991296));
#77130=CARTESIAN_POINT('Ctrl Pts',(-19.0945845827141,-16.8652518239961,
-2.49090477702753));
#77131=CARTESIAN_POINT('Ctrl Pts',(-19.0090766668656,-16.8526873990585,
-2.49579929498177));
#77132=CARTESIAN_POINT('Ctrl Pts',(-18.976279893557,-16.8486500167908,-2.49765037755845));
#77133=CARTESIAN_POINT('Ctrl Pts',(-18.7852284832504,-16.8296592150614,
-2.50831766663554));
#77134=CARTESIAN_POINT('Ctrl Pts',(-18.6257996033672,-16.8318011326506,
-2.51671730677738));
#77135=CARTESIAN_POINT('Ctrl Pts',(-18.4217059616401,-16.8576384862318,
-2.5281621761271));
#77136=CARTESIAN_POINT('Ctrl Pts',(-18.3755031033387,-16.8650507602765,
-2.53080323672204));
#77137=CARTESIAN_POINT('Ctrl Pts',(-18.3129815181106,-16.8772184166345,
-2.5344906560672));
#77138=CARTESIAN_POINT('Ctrl Pts',(-18.2964160470553,-16.8806488882883,
-2.53547864972362));
#77139=CARTESIAN_POINT('Ctrl Pts',(-18.2681428715129,-16.886858144027,-2.53718650104151));
#77140=CARTESIAN_POINT('Ctrl Pts',(-18.2564142548678,-16.8895389481557,
-2.53790137165594));
#77141=CARTESIAN_POINT('Ctrl Pts',(-18.2398024748614,-16.8934851850898,
-2.53892379564829));
#77142=CARTESIAN_POINT('Ctrl Pts',(-18.2348997548702,-16.8946683832762,
-2.53922677982418));
#77143=CARTESIAN_POINT('Ctrl Pts',(-18.2264687918622,-16.8967349801915,
-2.53975000037692));
#77144=CARTESIAN_POINT('Ctrl Pts',(-18.2229384733949,-16.8976099823181,
-2.53996975392649));
#77145=CARTESIAN_POINT('Ctrl Pts',(-18.2161063943996,-16.8993220380594,
-2.54039634791947));
#77146=CARTESIAN_POINT('Ctrl Pts',(-18.2128043905838,-16.9001579645345,
-2.54060311726895));
#77147=CARTESIAN_POINT('Ctrl Pts',(-18.2039189563164,-16.9024302097678,
-2.54116108719151));
#77148=CARTESIAN_POINT('Ctrl Pts',(-18.1983393998172,-16.9038813614615,
-2.5415131323691));
#77149=CARTESIAN_POINT('Ctrl Pts',(-18.1777566817011,-16.9093244500454,
-2.542817808868));
#77150=CARTESIAN_POINT('Ctrl Pts',(-18.1627920600465,-16.9134584898482,
-2.54377816205421));
#77151=CARTESIAN_POINT('Ctrl Pts',(-18.014865766124,-16.9560803968292,-2.55337931936512));
#77152=CARTESIAN_POINT('Ctrl Pts',(-17.8859477015773,-17.0073534823636,
-2.56259251617903));
#77153=CARTESIAN_POINT('Ctrl Pts',(-17.6236863361639,-17.1427291877668,
-2.58207676758641));
#77154=CARTESIAN_POINT('Ctrl Pts',(-17.4927956980432,-17.229883024082,-2.59224665750888));
#77155=CARTESIAN_POINT('Ctrl Pts',(-17.3584531866092,-17.342681320773,-2.60299063285758));
#77156=CARTESIAN_POINT('Ctrl Pts',(-17.3443525729114,-17.3548413634553,
-2.60412330254172));
#77157=CARTESIAN_POINT('Ctrl Pts',(-17.3240360895543,-17.3728346027039,
-2.60576305051107));
#77158=CARTESIAN_POINT('Ctrl Pts',(-17.3176924123458,-17.3785215599685,
-2.60627618129264));
#77159=CARTESIAN_POINT('Ctrl Pts',(-17.3066111321943,-17.3885769787169,
-2.60717459364726));
#77160=CARTESIAN_POINT('Ctrl Pts',(-17.3018588554306,-17.3929290372567,
-2.607560559442));
#77161=CARTESIAN_POINT('Ctrl Pts',(-17.2926555280229,-17.4014348846445,
-2.608309382641));
#77162=CARTESIAN_POINT('Ctrl Pts',(-17.2882023832658,-17.4055863048676,
-2.60867233520964));
#77163=CARTESIAN_POINT('Ctrl Pts',(-17.2775771800516,-17.4155776081885,
-2.60953988495517));
#77164=CARTESIAN_POINT('Ctrl Pts',(-17.271422219591,-17.4214355825454,-2.61004369956364));
#77165=CARTESIAN_POINT('Ctrl Pts',(-17.2492045896015,-17.4428375816475,
-2.61186711747284));
#77166=CARTESIAN_POINT('Ctrl Pts',(-17.2333527291824,-17.4585990356322,
-2.61317725984456));
#77167=CARTESIAN_POINT('Ctrl Pts',(-17.0899891072817,-17.6057331846057,
-2.62512213612595));
#77168=CARTESIAN_POINT('Ctrl Pts',(-16.9797754269409,-17.7528717634576,
-2.63492742701779));
#77169=CARTESIAN_POINT('Ctrl Pts',(-16.8496864969737,-17.9836282922652,
-2.6493606634437));
#77170=CARTESIAN_POINT('Ctrl Pts',(-16.8136801494142,-18.0571532449666,
-2.65385439815567));
#77171=CARTESIAN_POINT('Ctrl Pts',(-16.76790205596,-18.1662021164378,-2.66061627690045));
#77172=CARTESIAN_POINT('Ctrl Pts',(-16.7546560641544,-18.2001910733189,
-2.66273718358911));
#77173=CARTESIAN_POINT('Ctrl Pts',(-16.7397559652177,-18.2415523418886,
-2.66535332811062));
#77174=CARTESIAN_POINT('Ctrl Pts',(-16.7372539102181,-18.2486151876004,
-2.66580128276438));
#77175=CARTESIAN_POINT('Ctrl Pts',(-16.7334194712451,-18.2596244541528,
-2.66650165103914));
#77176=CARTESIAN_POINT('Ctrl Pts',(-16.7320611220711,-18.2635618569029,
-2.66675255321516));
#77177=CARTESIAN_POINT('Ctrl Pts',(-16.7295616245501,-18.270877022409,-2.66721951788925));
#77178=CARTESIAN_POINT('Ctrl Pts',(-16.7284173860902,-18.2742536685736,
-2.66743539468765));
#77179=CARTESIAN_POINT('Ctrl Pts',(-16.7258473618599,-18.2819013087203,
-2.66792506252116));
#77180=CARTESIAN_POINT('Ctrl Pts',(-16.7244266766088,-18.2861739482626,
-2.66819914837998));
#77181=CARTESIAN_POINT('Ctrl Pts',(-16.7201749544556,-18.2990983578693,
-2.66902972057012));
#77182=CARTESIAN_POINT('Ctrl Pts',(-16.7173861244278,-18.307763755766,-2.66958859654811));
#77183=CARTESIAN_POINT('Ctrl Pts',(-16.6964027866544,-18.3744342186201,
-2.67390241390562));
#77184=CARTESIAN_POINT('Ctrl Pts',(-16.6806602016957,-18.433175512017,-2.67778311973229));
#77185=CARTESIAN_POINT('Ctrl Pts',(-16.6544953518538,-18.5508495944172,
-2.68560931693323));
#77186=CARTESIAN_POINT('Ctrl Pts',(-16.6439997300583,-18.6097141394462,
-2.68954919806779));
#77187=CARTESIAN_POINT('Ctrl Pts',(-16.6214547373713,-18.776814584,-2.7006885988515));
#77188=CARTESIAN_POINT('Ctrl Pts',(-16.6152410173306,-18.8856579376055,
-2.70788290331176));
#77189=CARTESIAN_POINT('Ctrl Pts',(-16.6189294810739,-19.0693393875393,
-2.71968573748178));
#77190=CARTESIAN_POINT('Ctrl Pts',(-16.6244003470743,-19.1440501695098,
-2.72439467406062));
#77191=CARTESIAN_POINT('Ctrl Pts',(-16.6361815638864,-19.2369554518382,
-2.7301315167553));
#77192=CARTESIAN_POINT('Ctrl Pts',(-16.6387924334566,-19.2555573903308,
-2.73127433200432));
#77193=CARTESIAN_POINT('Ctrl Pts',(-16.6429515323512,-19.2825728436937,
-2.73292595535522));
#77194=CARTESIAN_POINT('Ctrl Pts',(-16.644303662991,-19.2910152230879,-2.73344094020871));
#77195=CARTESIAN_POINT('Ctrl Pts',(-16.6467652682766,-19.3058103417579,
-2.73434148848935));
#77196=CARTESIAN_POINT('Ctrl Pts',(-16.6478526870343,-19.3121665910108,
-2.73472774629328));
#77197=CARTESIAN_POINT('Ctrl Pts',(-16.6500215868135,-19.3245049348253,
-2.73547632877471));
#77198=CARTESIAN_POINT('Ctrl Pts',(-16.6510998235812,-19.3304875286672,
-2.73583875240774));
#77199=CARTESIAN_POINT('Ctrl Pts',(-16.653740677822,-19.3447871760181,-2.73670375035126));
#77200=CARTESIAN_POINT('Ctrl Pts',(-16.6553274331522,-19.3530997084849,
-2.73720555256272));
#77201=CARTESIAN_POINT('Ctrl Pts',(-16.6612435667179,-19.3831142283741,
-2.73901389463681));
#77202=CARTESIAN_POINT('Ctrl Pts',(-16.6658634084498,-19.4047579958013,
-2.7403111798372));
#77203=CARTESIAN_POINT('Ctrl Pts',(-16.712356256267,-19.6069881747458,-2.75237946205574));
#77204=CARTESIAN_POINT('Ctrl Pts',(-16.7774363137221,-19.7814079276443,
-2.76229617748199));
#77205=CARTESIAN_POINT('Ctrl Pts',(-16.9020687769329,-20.0160309433708,
-2.77677838677597));
#77206=CARTESIAN_POINT('Ctrl Pts',(-16.9437294307967,-20.0847237656925,
-2.78119283318351));
#77207=CARTESIAN_POINT('Ctrl Pts',(-17.0096109285556,-20.1806057863731,
-2.78784702134053));
#77208=CARTESIAN_POINT('Ctrl Pts',(-17.0307911844307,-20.2098033347825,
-2.78994486071768));
#77209=CARTESIAN_POINT('Ctrl Pts',(-17.0572437469074,-20.24437504082,-2.79253541732834));
#77210=CARTESIAN_POINT('Ctrl Pts',(-17.0618134287027,-20.250282267237,-2.79298192428639));
#77211=CARTESIAN_POINT('Ctrl Pts',(-17.0689768229347,-20.2594418242843,
-2.79368051603599));
#77212=CARTESIAN_POINT('Ctrl Pts',(-17.0715490783351,-20.262710966012,-2.79393110174537));
#77213=CARTESIAN_POINT('Ctrl Pts',(-17.0763441711972,-20.2687683427906,
-2.79439778391963));
#77214=CARTESIAN_POINT('Ctrl Pts',(-17.0785644240464,-20.2715585506529,
-2.79461369662171));
#77215=CARTESIAN_POINT('Ctrl Pts',(-17.0836087264691,-20.2778649943719,
-2.79510384257887));
#77216=CARTESIAN_POINT('Ctrl Pts',(-17.0864369547359,-20.2813778056135,
-2.79537837313561));
#77217=CARTESIAN_POINT('Ctrl Pts',(-17.0937678546657,-20.2904238493259,
-2.79608918027847));
#77218=CARTESIAN_POINT('Ctrl Pts',(-17.0982872670438,-20.2959433555661,
-2.79652662278851));
#77219=CARTESIAN_POINT('Ctrl Pts',(-17.1262020155252,-20.3296859324566,
-2.79922333626872));
#77220=CARTESIAN_POINT('Ctrl Pts',(-17.1502977877338,-20.3573184041027,
-2.80152877697819));
#77221=CARTESIAN_POINT('Ctrl Pts',(-17.2905198459883,-20.5099338860497,
-2.81475506622014));
#77222=CARTESIAN_POINT('Ctrl Pts',(-17.4207027263043,-20.6211453908159,
-2.82626658314038));
#77223=CARTESIAN_POINT('Ctrl Pts',(-17.6422309411859,-20.7682641858778,
-2.84354790066166));
#77224=CARTESIAN_POINT('Ctrl Pts',(-17.7251161516467,-20.8155806649673,
-2.84960399158042));
#77225=CARTESIAN_POINT('Ctrl Pts',(-17.8301635393875,-20.8664779788826,
-2.85677403699184));
#77226=CARTESIAN_POINT('Ctrl Pts',(-17.8495484397734,-20.8755102727644,
-2.85807747242254));
#77227=CARTESIAN_POINT('Ctrl Pts',(-17.8772897908168,-20.8879281420314,
-2.85991560516654));
#77228=CARTESIAN_POINT('Ctrl Pts',(-17.8855356458991,-20.8915562372278,
-2.86045860440219));
#77229=CARTESIAN_POINT('Ctrl Pts',(-17.8997946371104,-20.8977217176929,
-2.86139185880284));
#77230=CARTESIAN_POINT('Ctrl Pts',(-17.9057967607741,-20.900284113314,-2.8617829644363));
#77231=CARTESIAN_POINT('Ctrl Pts',(-17.9173074120821,-20.9051353761622,
-2.86252973492477));
#77232=CARTESIAN_POINT('Ctrl Pts',(-17.9228139434107,-20.9074287927441,
-2.86288555160323));
#77233=CARTESIAN_POINT('Ctrl Pts',(-17.9371485581939,-20.91332804874,-2.86380815248949));
#77234=CARTESIAN_POINT('Ctrl Pts',(-17.9459915056895,-20.9168975933875,
-2.8643737045856));
#77235=CARTESIAN_POINT('Ctrl Pts',(-17.9761783563008,-20.928846254373,-2.86629235026561));
#77236=CARTESIAN_POINT('Ctrl Pts',(-17.9976346070627,-20.9369384941645,
-2.86763581300588));
#77237=CARTESIAN_POINT('Ctrl Pts',(-18.1851701243143,-21.0042081119377,
-2.87921379355666));
#77238=CARTESIAN_POINT('Ctrl Pts',(-18.3579047976642,-21.0427729255352,
-2.88868917458312));
#77239=CARTESIAN_POINT('Ctrl Pts',(-18.6194739823872,-21.0676659669617,
-2.90298760447507));
#77240=CARTESIAN_POINT('Ctrl Pts',(-18.7059267822595,-21.0705769340084,
-2.9077208684055));
#77241=CARTESIAN_POINT('Ctrl Pts',(-18.8299702073384,-21.0671591569455,
-2.91480681872399));
#77242=CARTESIAN_POINT('Ctrl Pts',(-18.8675956958097,-21.065116261605,-2.91699559974952));
#77243=CARTESIAN_POINT('Ctrl Pts',(-18.9126825053349,-21.0614593540092,
-2.91968700219917));
#77244=CARTESIAN_POINT('Ctrl Pts',(-18.9202176178737,-21.0608075300537,
-2.92013910931319));
#77245=CARTESIAN_POINT('Ctrl Pts',(-18.9319118510765,-21.0597327571016,
-2.92084457189483));
#77246=CARTESIAN_POINT('Ctrl Pts',(-18.9360735719884,-21.0593378340849,
-2.9210963802099));
#77247=CARTESIAN_POINT('Ctrl Pts',(-18.9437810432223,-21.0585833986757,
-2.92156416115829));
#77248=CARTESIAN_POINT('Ctrl Pts',(-18.9473270656625,-21.0582272584276,
-2.92177994256916));
#77249=CARTESIAN_POINT('Ctrl Pts',(-18.9553310718424,-21.0574029660065,
-2.92226827503101));
#77250=CARTESIAN_POINT('Ctrl Pts',(-18.9597884524445,-21.056929610823,-2.92254111395026));
#77251=CARTESIAN_POINT('Ctrl Pts',(-18.9729092891475,-21.0554940773037,
-2.9233468012166));
#77252=CARTESIAN_POINT('Ctrl Pts',(-18.9815682219235,-21.0544925567489,
-2.92388178430716));
#77253=CARTESIAN_POINT('Ctrl Pts',(-19.0431247851564,-21.0469871916588,
-2.92770715323812));
#77254=CARTESIAN_POINT('Ctrl Pts',(-19.0957619578154,-21.0385418084244,
-2.93109442716222));
#77255=CARTESIAN_POINT('Ctrl Pts',(-19.165639585287,-21.0246068341795,-2.93569932437968));
#77256=CARTESIAN_POINT('Ctrl Pts',(-19.183214058549,-21.0208688998034,-2.93686677563015));
#77257=CARTESIAN_POINT('Ctrl Pts',(-19.2477667355174,-21.0062778284428,
-2.94118471749289));
#77258=CARTESIAN_POINT('Ctrl Pts',(-19.2944169913585,-20.9940446170198,
-2.94436322108441));
#77259=CARTESIAN_POINT('Ctrl Pts',(-19.4454006226561,-20.9488880873146,
-2.95477330183771));
#77260=CARTESIAN_POINT('Ctrl Pts',(-19.5476151913201,-20.909469454547,-2.96200586331425));
#77261=CARTESIAN_POINT('Ctrl Pts',(-19.7146198451544,-20.8297115769728,
-2.97390182191414));
#77262=CARTESIAN_POINT('Ctrl Pts',(-19.7811168240447,-20.7934571956495,
-2.9786646070532));
#77263=CARTESIAN_POINT('Ctrl Pts',(-19.8616163856955,-20.7437944328501,
-2.98445954348771));
#77264=CARTESIAN_POINT('Ctrl Pts',(-19.8775638003171,-20.7336587422455,
-2.98560923791801));
#77265=CARTESIAN_POINT('Ctrl Pts',(-19.9005446269231,-20.7186171297813,
-2.9872689067531));
#77266=CARTESIAN_POINT('Ctrl Pts',(-19.907686968211,-20.7138800622817,-2.98778514283673));
#77267=CARTESIAN_POINT('Ctrl Pts',(-19.9201552917799,-20.7055011399917,
-2.98868713489284));
#77268=CARTESIAN_POINT('Ctrl Pts',(-19.9254937215573,-20.7018780920649,
-2.98907359210613));
#77269=CARTESIAN_POINT('Ctrl Pts',(-19.9358248392117,-20.6947974454344,
-2.98982202182923));
#77270=CARTESIAN_POINT('Ctrl Pts',(-19.9408193702581,-20.6913426599469,
-2.9901840958295));
#77271=CARTESIAN_POINT('Ctrl Pts',(-19.9527192190574,-20.6830354394547,
-2.99104740250487));
#77272=CARTESIAN_POINT('Ctrl Pts',(-19.9596105557258,-20.6781630851042,
-2.99154787000295));
#77273=CARTESIAN_POINT('Ctrl Pts',(-19.9843472197686,-20.6604508010163,
-2.99334636737155));
#77274=CARTESIAN_POINT('Ctrl Pts',(-20.0020218091838,-20.6473740160565,
-2.99463527563848));
#77275=CARTESIAN_POINT('Ctrl Pts',(-20.1679063249765,-20.5205964570162,
-3.00677962427125));
#77276=CARTESIAN_POINT('Ctrl Pts',(-20.3006543344855,-20.3880300454364,
-3.01676515693063));
#77277=CARTESIAN_POINT('Ctrl Pts',(-20.462557625633,-20.1767749022675,-3.03127852268068));
#77278=CARTESIAN_POINT('Ctrl Pts',(-20.5072414949363,-20.1111366026836,
-3.03564445976581));
#77279=CARTESIAN_POINT('Ctrl Pts',(-20.5665926592175,-20.0124602166786,
-3.04223265684119));
#77280=CARTESIAN_POINT('Ctrl Pts',(-20.5842695945084,-19.9813074422148,
-3.04431623325168));
#77281=CARTESIAN_POINT('Ctrl Pts',(-20.604659326247,-19.9431499558446,-3.04689096520608));
#77282=CARTESIAN_POINT('Ctrl Pts',(-20.6081371447691,-19.9365580270833,
-3.04733656748382));
#77283=CARTESIAN_POINT('Ctrl Pts',(-20.6135001055998,-19.9262615815686,
-3.04803404893226));
#77284=CARTESIAN_POINT('Ctrl Pts',(-20.6154093082858,-19.9225695700379,
-3.04828443672385));
#77285=CARTESIAN_POINT('Ctrl Pts',(-20.618936353984,-19.9156994651866,-3.04875094291312));
#77286=CARTESIAN_POINT('Ctrl Pts',(-20.6205570438794,-19.9125228978802,
-3.04896687876149));
#77287=CARTESIAN_POINT('Ctrl Pts',(-20.6242111978435,-19.9053157963717,
-3.04945732687813));
#77288=CARTESIAN_POINT('Ctrl Pts',(-20.6262397902928,-19.9012828636525,
-3.04973213801056));
#77289=CARTESIAN_POINT('Ctrl Pts',(-20.6322139769686,-19.8893106729462,
-3.05054896180295));
#77290=CARTESIAN_POINT('Ctrl Pts',(-20.6361225578581,-19.8813531990358,
-3.05109319647717));
#77291=CARTESIAN_POINT('Ctrl Pts',(-20.6648568363037,-19.8219124810826,
-3.05516702627434));
#77292=CARTESIAN_POINT('Ctrl Pts',(-20.6876362395481,-19.7694717412689,
-3.05880796392093));
#77293=CARTESIAN_POINT('Ctrl Pts',(-20.7131593808188,-19.703532466891,-3.06338860271513));
#77294=CARTESIAN_POINT('Ctrl Pts',(-20.7179316577104,-19.6908422631791,
-3.06427030004251));
#77295=CARTESIAN_POINT('Ctrl Pts',(-20.7225805657411,-19.6781104141636,
-3.06515450115675));
#77296=CARTESIAN_POINT('',(-20.8479141126547,-18.952828455763,-2.0890042932752));
#77297=CARTESIAN_POINT('Ctrl Pts',(-20.7202230519095,-19.6772708889146,
-2.84456322442383));
#77298=CARTESIAN_POINT('Ctrl Pts',(-20.6328469601815,-19.9216249165611,
-2.82899806527974));
#77299=CARTESIAN_POINT('Ctrl Pts',(-20.1480308925685,-20.7713282564288,
-2.77104097057519));
#77300=CARTESIAN_POINT('Ctrl Pts',(-18.3741968385222,-21.4292710094645,
-2.67069194031011));
#77301=CARTESIAN_POINT('Ctrl Pts',(-16.4562524857842,-19.9903623098931,
-2.54351613362868));
#77302=CARTESIAN_POINT('Ctrl Pts',(-16.6280001024638,-17.5988205946497,
-2.41634032694725));
#77303=CARTESIAN_POINT('Ctrl Pts',(-18.7318719157381,-16.448737081536,-2.28916452026583));
#77304=CARTESIAN_POINT('Ctrl Pts',(-20.5383021468591,-17.4322383264222,
-2.18006983762423));
#77305=CARTESIAN_POINT('Ctrl Pts',(-20.8463943934263,-18.5471996728808,
-2.11336709054313));
#77306=CARTESIAN_POINT('Ctrl Pts',(-20.8478239065824,-18.9528314138757,
-2.0890562790225));
#77307=CARTESIAN_POINT('Ctrl Pts',(-20.8509998750793,-18.9527272648688,
-2.08722596880618));
#77308=CARTESIAN_POINT('Ctrl Pts',(-20.8509329970117,-19.1474030521012,
-2.07601660755437));
#77309=CARTESIAN_POINT('Ctrl Pts',(-20.8240164192313,-19.3411372216795,
-2.0657352891835));
#77310=CARTESIAN_POINT('Ctrl Pts',(-20.7567161848195,-19.5789442372845,
-2.05215238229222));
#77311=CARTESIAN_POINT('Ctrl Pts',(-20.7405652872149,-19.6288561003616,
-2.04923741397087));
#77312=CARTESIAN_POINT('Ctrl Pts',(-20.7225805826894,-19.6781103677477,
-2.04625070052543));
#77313=CARTESIAN_POINT('Origin',(-18.734,-18.952,0.));
#77314=CARTESIAN_POINT('',(-20.7225806439552,-19.6781101999605,-1.24458624895941));
#77315=CARTESIAN_POINT('',(-20.7225805819607,-19.6781103697435,-1.46829802089257));
#77316=CARTESIAN_POINT('',(-20.7225805821191,-19.6781103693095,0.));
#77317=CARTESIAN_POINT('Ctrl Pts',(-20.7225805819607,-19.6781103697434,
-1.46829802089257));
#77318=CARTESIAN_POINT('Ctrl Pts',(-20.7720931560047,-19.5425115029463,
-1.47674759264403));
#77319=CARTESIAN_POINT('Ctrl Pts',(-20.8076106549703,-19.4021955091639,
-1.48469159119666));
#77320=CARTESIAN_POINT('Ctrl Pts',(-20.8435716231799,-19.1571126846671,
-1.4981609862824));
#77321=CARTESIAN_POINT('Ctrl Pts',(-20.8510665767008,-19.0539337997499,
-1.50372418439499));
#77322=CARTESIAN_POINT('Ctrl Pts',(-20.8509605931235,-18.8905719691387,
-1.51286258178651));
#77323=CARTESIAN_POINT('Ctrl Pts',(-20.8483662197456,-18.8305518846646,
-1.51629231097292));
#77324=CARTESIAN_POINT('Ctrl Pts',(-20.8424571653604,-18.7617954033505,
-1.52038555277385));
#77325=CARTESIAN_POINT('Ctrl Pts',(-20.8416326174778,-18.7528665018886,
-1.52092031606078));
#77326=CARTESIAN_POINT('Ctrl Pts',(-20.8403055944572,-18.7394292637794,
-1.52173027738312));
#77327=CARTESIAN_POINT('Ctrl Pts',(-20.8398453004456,-18.7349167329088,
-1.52200316307499));
#77328=CARTESIAN_POINT('Ctrl Pts',(-20.8389970510928,-18.7268575017177,
-1.52249215995441));
#77329=CARTESIAN_POINT('Ctrl Pts',(-20.8386146291968,-18.7233102714294,
-1.52270795724757));
#77330=CARTESIAN_POINT('Ctrl Pts',(-20.8377689773509,-18.715648065319,-1.52317533193935));
#77331=CARTESIAN_POINT('Ctrl Pts',(-20.8373026471316,-18.7115335345996,
-1.52342707634132));
#77332=CARTESIAN_POINT('Ctrl Pts',(-20.8359714183482,-18.700088014928,-1.52412945106569));
#77333=CARTESIAN_POINT('Ctrl Pts',(-20.8350802524046,-18.6927602248131,
-1.52458152096667));
#77334=CARTESIAN_POINT('Ctrl Pts',(-20.8297855243033,-18.6510449721524,
-1.52716806677283));
#77335=CARTESIAN_POINT('Ctrl Pts',(-20.8245763700799,-18.6167672271824,
-1.52934386967377));
#77336=CARTESIAN_POINT('Ctrl Pts',(-20.805407203348,-18.5085850836545,-1.53633896031892));
#77337=CARTESIAN_POINT('Ctrl Pts',(-20.7883503689925,-18.4352915707807,
-1.5412675751516));
#77338=CARTESIAN_POINT('Ctrl Pts',(-20.7136651896318,-18.1774233514788,
-1.55897631652309));
#77339=CARTESIAN_POINT('Ctrl Pts',(-20.6347145051753,-17.9999712102452,
-1.57174497002659));
#77340=CARTESIAN_POINT('Ctrl Pts',(-20.5215596546255,-17.8176409598084,
-1.58493005964286));
#77341=CARTESIAN_POINT('Ctrl Pts',(-20.5100907444826,-17.7997666599859,
-1.5862249121803));
#77342=CARTESIAN_POINT('Ctrl Pts',(-20.4937578044299,-17.7751352437741,
-1.58801303729796));
#77343=CARTESIAN_POINT('Ctrl Pts',(-20.4891202512924,-17.7682301358412,
-1.58851473814774));
#77344=CARTESIAN_POINT('Ctrl Pts',(-20.4810444540192,-17.7563574238619,
-1.58937815825898));
#77345=CARTESIAN_POINT('Ctrl Pts',(-20.4776254463123,-17.7513769124568,
-1.58974059901217));
#77346=CARTESIAN_POINT('Ctrl Pts',(-20.4705005725153,-17.7410926446403,
-1.59048953820632));
#77347=CARTESIAN_POINT('Ctrl Pts',(-20.4667916131035,-17.7357910999329,
-1.59087591362798));
#77348=CARTESIAN_POINT('Ctrl Pts',(-20.4580471971384,-17.7234131324265,
-1.59177876182168));
#77349=CARTESIAN_POINT('Ctrl Pts',(-20.4529923593877,-17.716350494303,-1.59229448462309));
#77350=CARTESIAN_POINT('Ctrl Pts',(-20.4364321359028,-17.6935107857039,
-1.5939643184017));
#77351=CARTESIAN_POINT('Ctrl Pts',(-20.4247516920709,-17.6778614544143,
-1.59511164885719));
#77352=CARTESIAN_POINT('Ctrl Pts',(-20.3638543848995,-17.5985842527767,
-1.6009440987315));
#77353=CARTESIAN_POINT('Ctrl Pts',(-20.3112537720283,-17.537633684328,-1.60549259413782));
#77354=CARTESIAN_POINT('Ctrl Pts',(-20.1384828374626,-17.3590974186498,
-1.61926744787057));
#77355=CARTESIAN_POINT('Ctrl Pts',(-20.0077162434858,-17.2527206740547,
-1.62810931945867));
#77356=CARTESIAN_POINT('Ctrl Pts',(-19.8645504722943,-17.1621545623342,
-1.63762197913388));
#77357=CARTESIAN_POINT('Ctrl Pts',(-19.8633364114307,-17.1613882802404,
-1.63770263978496));
#77358=CARTESIAN_POINT('Ctrl Pts',(-19.8165501446093,-17.1319245750012,
-1.6408107992702));
#77359=CARTESIAN_POINT('Ctrl Pts',(-19.769904206213,-17.1049778566222,-1.64389995115153));
#77360=CARTESIAN_POINT('Ctrl Pts',(-19.7145580901597,-17.0757614222467,
-1.64761374906773));
#77361=CARTESIAN_POINT('Ctrl Pts',(-19.7068048260349,-17.071729771199,-1.64813508316971));
#77362=CARTESIAN_POINT('Ctrl Pts',(-19.6950330254656,-17.0657008032327,
-1.64892859080482));
#77363=CARTESIAN_POINT('Ctrl Pts',(-19.6910326250181,-17.0636680139448,
-1.64919858901596));
#77364=CARTESIAN_POINT('Ctrl Pts',(-19.6838431557468,-17.0600434245146,
-1.64968449156431));
#77365=CARTESIAN_POINT('Ctrl Pts',(-19.680656505283,-17.0584469469397,-1.6499000984515));
#77366=CARTESIAN_POINT('Ctrl Pts',(-19.6737267013854,-17.0549970552061,
-1.65036948900504));
#77367=CARTESIAN_POINT('Ctrl Pts',(-19.6699821394481,-17.0531466934511,
-1.65062345280078));
#77368=CARTESIAN_POINT('Ctrl Pts',(-19.65945663646,-17.0479842528489,-1.65133817465765));
#77369=CARTESIAN_POINT('Ctrl Pts',(-19.6526635046141,-17.0446973725394,
-1.65180045401116));
#77370=CARTESIAN_POINT('Ctrl Pts',(-19.6121122934695,-17.0253434237479,
-1.65456529495592));
#77371=CARTESIAN_POINT('Ctrl Pts',(-19.5779531778002,-17.010137646603,-1.6569159911075));
#77372=CARTESIAN_POINT('Ctrl Pts',(-19.4646002505116,-16.9632348036155,
-1.66474517783172));
#77373=CARTESIAN_POINT('Ctrl Pts',(-19.3838947010915,-16.935419047224,-1.67036146853556));
#77374=CARTESIAN_POINT('Ctrl Pts',(-19.1303439587519,-16.8648362097004,
-1.68774849196257));
#77375=CARTESIAN_POINT('Ctrl Pts',(-18.9535825726714,-16.8389100513405,
-1.69943933765766));
#77376=CARTESIAN_POINT('Ctrl Pts',(-18.7528413217338,-16.8349610585024,
-1.71179541625068));
#77377=CARTESIAN_POINT('Ctrl Pts',(-18.7300385391062,-16.8348809089096,
-1.71318715496088));
#77378=CARTESIAN_POINT('Ctrl Pts',(-18.6977241054554,-16.8352894407271,
-1.71514335073775));
#77379=CARTESIAN_POINT('Ctrl Pts',(-18.6882108216452,-16.8354738631353,
-1.71571727820927));
#77380=CARTESIAN_POINT('Ctrl Pts',(-18.6727398788415,-16.8358781385027,
-1.71664750104682));
#77381=CARTESIAN_POINT('Ctrl Pts',(-18.6667814139094,-16.8360590277692,
-1.71700501229205));
#77382=CARTESIAN_POINT('Ctrl Pts',(-18.6542981447292,-16.8364907826573,
-1.71775246541144));
#77383=CARTESIAN_POINT('Ctrl Pts',(-18.6477735683102,-16.8367466727726,
-1.71814224583394));
#77384=CARTESIAN_POINT('Ctrl Pts',(-18.6322317703546,-16.8374282428006,
-1.71906865220709));
#77385=CARTESIAN_POINT('Ctrl Pts',(-18.6232158351792,-16.8378814220628,
-1.71960441083953));
#77386=CARTESIAN_POINT('Ctrl Pts',(-18.5927430277503,-16.8396085883,-1.72140981157502));
#77387=CARTESIAN_POINT('Ctrl Pts',(-18.5713023058927,-16.8411517063428,
-1.7226710194346));
#77388=CARTESIAN_POINT('Ctrl Pts',(-18.3711113374509,-16.8586281824042,
-1.7343712045856));
#77389=CARTESIAN_POINT('Ctrl Pts',(-18.1950470064643,-16.8969013635447,
-1.74401336695471));
#77390=CARTESIAN_POINT('Ctrl Pts',(-17.9123555806182,-16.9972345763578,
-1.76033857027388));
#77391=CARTESIAN_POINT('Ctrl Pts',(-17.8024670832392,-17.0471521413233,
-1.76694910621919));
#77392=CARTESIAN_POINT('Ctrl Pts',(-17.689157312473,-17.1107822137987,-1.77465096526347));
#77393=CARTESIAN_POINT('Ctrl Pts',(-17.6809088778169,-17.1154874738563,
-1.77521700333436));
#77394=CARTESIAN_POINT('Ctrl Pts',(-17.6687290579812,-17.1225443971041,
-1.77606125136031));
#77395=CARTESIAN_POINT('Ctrl Pts',(-17.6647730693753,-17.1248536586254,
-1.77633678946594));
#77396=CARTESIAN_POINT('Ctrl Pts',(-17.657745774603,-17.1289863960063,-1.77682867067709));
#77397=CARTESIAN_POINT('Ctrl Pts',(-17.6546715578725,-17.1308048232506,
-1.7770446848463));
#77398=CARTESIAN_POINT('Ctrl Pts',(-17.6480695597411,-17.1347325533149,
-1.77751039119574));
#77399=CARTESIAN_POINT('Ctrl Pts',(-17.6445433666054,-17.136844321511,-1.77776023901127));
#77400=CARTESIAN_POINT('Ctrl Pts',(-17.6348212205239,-17.1427052597282,
-1.77845212054551));
#77401=CARTESIAN_POINT('Ctrl Pts',(-17.628638389739,-17.1464759338364,-1.77889552601222));
#77402=CARTESIAN_POINT('Ctrl Pts',(-17.5947783719678,-17.1673649810112,
-1.78134203262665));
#77403=CARTESIAN_POINT('Ctrl Pts',(-17.5674810060627,-17.1850870886606,
-1.78338149012634));
#77404=CARTESIAN_POINT('Ctrl Pts',(-17.4062222837481,-17.2951458252544,
-1.79578761632431));
#77405=CARTESIAN_POINT('Ctrl Pts',(-17.2828639885251,-17.4020439918414,
-1.80674408137016));
#77406=CARTESIAN_POINT('Ctrl Pts',(-17.0940640645746,-17.6081460680513,
-1.82500120375695));
#77407=CARTESIAN_POINT('Ctrl Pts',(-17.0224165578849,-17.7006714304132,
-1.83244184753139));
#77408=CARTESIAN_POINT('Ctrl Pts',(-16.9509757340412,-17.8106334283907,
-1.84044872018204));
#77409=CARTESIAN_POINT('Ctrl Pts',(-16.9433122522029,-17.8226946429811,
-1.84131669273718));
#77410=CARTESIAN_POINT('Ctrl Pts',(-16.9313097879687,-17.842014199276,-1.84269099629933));
#77411=CARTESIAN_POINT('Ctrl Pts',(-16.9268912599426,-17.8492223781695,
-1.84320025535469));
#77412=CARTESIAN_POINT('Ctrl Pts',(-16.9191746503873,-17.8619818169293,
-1.8440956310349));
#77413=CARTESIAN_POINT('Ctrl Pts',(-16.9158585847764,-17.8675220220293,
-1.84448240378293));
#77414=CARTESIAN_POINT('Ctrl Pts',(-16.909052320419,-17.8790123254048,-1.84528047090647));
#77415=CARTESIAN_POINT('Ctrl Pts',(-16.9055657493798,-17.8849644917192,
-1.84569162990037));
#77416=CARTESIAN_POINT('Ctrl Pts',(-16.8966908776356,-17.9002866285896,
-1.84674433828627));
#77417=CARTESIAN_POINT('Ctrl Pts',(-16.8913450888508,-17.9096810892519,
-1.84738434637507));
#77418=CARTESIAN_POINT('Ctrl Pts',(-16.8693339283149,-17.9490611758034,
-1.85004501217718));
#77419=CARTESIAN_POINT('Ctrl Pts',(-16.8533261471882,-17.9794096957476,
-1.85204214106567));
#77420=CARTESIAN_POINT('Ctrl Pts',(-16.8135457661922,-18.0594860747149,
-1.85718622303641));
#77421=CARTESIAN_POINT('Ctrl Pts',(-16.7909643176087,-18.1097776105255,
-1.86029378691145));
#77422=CARTESIAN_POINT('Ctrl Pts',(-16.7295080505817,-18.2623206019634,
-1.86943820421793));
#77423=CARTESIAN_POINT('Ctrl Pts',(-16.6965647403786,-18.3667615068895,
-1.87532632806816));
#77424=CARTESIAN_POINT('Ctrl Pts',(-16.6614948457228,-18.5178305125628,
-1.88376987107214));
#77425=CARTESIAN_POINT('Ctrl Pts',(-16.6525992748352,-18.5627037860073,
-1.88627060963726));
#77426=CARTESIAN_POINT('Ctrl Pts',(-16.6414615163854,-18.6303007519883,
-1.89006945553716));
#77427=CARTESIAN_POINT('Ctrl Pts',(-16.6381218045566,-18.6528307339971,
-1.89134087530487));
#77428=CARTESIAN_POINT('Ctrl Pts',(-16.6350173565239,-18.6763882500269,
-1.89267965899724));
#77429=CARTESIAN_POINT('Ctrl Pts',(-16.6348890764467,-18.6773669631099,
-1.89273529654612));
#77430=CARTESIAN_POINT('Ctrl Pts',(-16.6324974615984,-18.6957133628997,
-1.89377856834965));
#77431=CARTESIAN_POINT('Ctrl Pts',(-16.6304491159064,-18.7131079602769,
-1.89477311962891));
#77432=CARTESIAN_POINT('Ctrl Pts',(-16.6250305537704,-18.7646179557352,
-1.89773935511748));
#77433=CARTESIAN_POINT('Ctrl Pts',(-16.6222730658847,-18.7987903068576,
-1.89973448825879));
#77434=CARTESIAN_POINT('Ctrl Pts',(-16.6199541902419,-18.8399819454601,
-1.90218822447091));
#77435=CARTESIAN_POINT('Ctrl Pts',(-16.619596315564,-18.8469534080429,-1.9026051854378));
#77436=CARTESIAN_POINT('Ctrl Pts',(-16.6190661743308,-18.8583846602077,
-1.90329182261017));
#77437=CARTESIAN_POINT('Ctrl Pts',(-16.6188735170734,-18.8628435129217,
-1.90356038335881));
#77438=CARTESIAN_POINT('Ctrl Pts',(-16.6185524253135,-18.8708627600133,
-1.90404475977978));
#77439=CARTESIAN_POINT('Ctrl Pts',(-16.6184188776031,-18.8744228950945,
-1.90426028618967));
#77440=CARTESIAN_POINT('Ctrl Pts',(-16.6181476248048,-18.8821764398172,
-1.90473075032974));
#77441=CARTESIAN_POINT('Ctrl Pts',(-16.6180134005704,-18.8863698734934,
-1.90498587502555));
#77442=CARTESIAN_POINT('Ctrl Pts',(-16.6176701236929,-18.8981936700985,
-1.90570708368143));
#77443=CARTESIAN_POINT('Ctrl Pts',(-16.6174898759185,-18.905824713597,-1.90617473268144));
#77444=CARTESIAN_POINT('Ctrl Pts',(-16.6166422978356,-18.9523701010658,
-1.9090397744387));
#77445=CARTESIAN_POINT('Ctrl Pts',(-16.6170069957211,-18.991293154584,-1.91148936322848));
#77446=CARTESIAN_POINT('Ctrl Pts',(-16.624432178869,-19.192216446517,-1.92433805849365));
#77447=CARTESIAN_POINT('Ctrl Pts',(-16.6490153671944,-19.3530249496497,
-1.93525759681636));
#77448=CARTESIAN_POINT('Ctrl Pts',(-16.720801572638,-19.6160210132374,-1.95302136151426));
#77449=CARTESIAN_POINT('Ctrl Pts',(-16.7581895162412,-19.7201610518911,
-1.96004026467851));
#77450=CARTESIAN_POINT('Ctrl Pts',(-16.809364870051,-19.8338558992318,-1.9676522676726));
#77451=CARTESIAN_POINT('Ctrl Pts',(-16.8153170027438,-19.8467322403145,
-1.96851381223093));
#77452=CARTESIAN_POINT('Ctrl Pts',(-16.8250096346055,-19.8671588670269,
-1.96987989211645));
#77453=CARTESIAN_POINT('Ctrl Pts',(-16.828666484445,-19.8747481589113,-1.97038730120075));
#77454=CARTESIAN_POINT('Ctrl Pts',(-16.8352038190521,-19.888110938308,-1.97128052825651));
#77455=CARTESIAN_POINT('Ctrl Pts',(-16.8380655604922,-19.8938934271563,
-1.9716669924283));
#77456=CARTESIAN_POINT('Ctrl Pts',(-16.8440471794529,-19.9058422781841,
-1.97246548443794));
#77457=CARTESIAN_POINT('Ctrl Pts',(-16.8471709088992,-19.9120066344886,
-1.97287737165393));
#77458=CARTESIAN_POINT('Ctrl Pts',(-16.8552835589183,-19.9278235453769,
-1.97393415242114));
#77459=CARTESIAN_POINT('Ctrl Pts',(-16.8603167474348,-19.9374532629306,
-1.97457748121119));
#77460=CARTESIAN_POINT('Ctrl Pts',(-16.8817820617469,-19.9777626112148,
-1.97727060546021));
#77461=CARTESIAN_POINT('Ctrl Pts',(-16.8988958476915,-20.008074419974,-1.97929613321528));
#77462=CARTESIAN_POINT('Ctrl Pts',(-16.9455837646253,-20.0862027630167,
-1.98453016001506));
#77463=CARTESIAN_POINT('Ctrl Pts',(-16.9763291082887,-20.1332883872032,
-1.98769743867443));
#77464=CARTESIAN_POINT('Ctrl Pts',(-17.0817706984249,-20.2815209961167,
-1.9978032875194));
#77465=CARTESIAN_POINT('Ctrl Pts',(-17.1636028273967,-20.3772510786442,
-2.00452990898683));
#77466=CARTESIAN_POINT('Ctrl Pts',(-17.3250192108307,-20.5351897250686,
-2.01688751694712));
#77467=CARTESIAN_POINT('Ctrl Pts',(-17.401463959395,-20.6000470132183,-2.02245412321344));
#77468=CARTESIAN_POINT('Ctrl Pts',(-17.4900160570699,-20.6649760445418,
-2.02895946080841));
#77469=CARTESIAN_POINT('Ctrl Pts',(-17.4978730895972,-20.6706544832367,
-2.02953715294625));
#77470=CARTESIAN_POINT('Ctrl Pts',(-17.5095311331976,-20.6789586946519,
-2.03039548033192));
#77471=CARTESIAN_POINT('Ctrl Pts',(-17.5133023117823,-20.681626402393,-2.03067331277748));
#77472=CARTESIAN_POINT('Ctrl Pts',(-17.5200080570562,-20.6863371495187,
-2.03116771579227));
#77473=CARTESIAN_POINT('Ctrl Pts',(-17.5229391003863,-20.6883851194223,
-2.03138394443113));
#77474=CARTESIAN_POINT('Ctrl Pts',(-17.5292300518527,-20.6927570368103,
-2.03184833071061));
#77475=CARTESIAN_POINT('Ctrl Pts',(-17.5325914517094,-20.6950786524439,
-2.03209663463902));
#77476=CARTESIAN_POINT('Ctrl Pts',(-17.5418367574082,-20.7014246538077,
-2.03278000064794));
#77477=CARTESIAN_POINT('Ctrl Pts',(-17.5477342403474,-20.7054290292111,
-2.03321638046797));
#77478=CARTESIAN_POINT('Ctrl Pts',(-17.5793268591596,-20.7266479998233,
-2.03555605303473));
#77479=CARTESIAN_POINT('Ctrl Pts',(-17.6053752782282,-20.7433267679299,
-2.03749213161147));
#77480=CARTESIAN_POINT('Ctrl Pts',(-17.6853208634728,-20.7920799048843,
-2.04343315903331));
#77481=CARTESIAN_POINT('Ctrl Pts',(-17.7402846192009,-20.8223343632513,
-2.04751558425808));
#77482=CARTESIAN_POINT('Ctrl Pts',(-17.9269437673714,-20.9145274204903,
-2.06119652295239));
#77483=CARTESIAN_POINT('Ctrl Pts',(-18.0636913134972,-20.9653423845116,
-2.07089652908973));
#77484=CARTESIAN_POINT('Ctrl Pts',(-18.2773306865386,-21.020523315321,-2.08502433209331));
#77485=CARTESIAN_POINT('Ctrl Pts',(-18.3510416139255,-21.0354300157609,
-2.08973101563419));
#77486=CARTESIAN_POINT('Ctrl Pts',(-18.4383920181184,-21.0483008988569,
-2.095113975572));
#77487=CARTESIAN_POINT('Ctrl Pts',(-18.4514048216643,-21.0500947344908,
-2.09591096010546));
#77488=CARTESIAN_POINT('Ctrl Pts',(-18.4725698737199,-21.0528118852477,
-2.09719942659657));
#77489=CARTESIAN_POINT('Ctrl Pts',(-18.4807121246604,-21.0538091120003,
-2.09769323066074));
#77490=CARTESIAN_POINT('Ctrl Pts',(-18.4952174439366,-21.0555001441856,
-2.09856966623564));
#77491=CARTESIAN_POINT('Ctrl Pts',(-18.5015782129253,-21.0562124607454,
-2.09895287706902));
#77492=CARTESIAN_POINT('Ctrl Pts',(-18.5149835319341,-21.0576521411115,
-2.09975817978));
#77493=CARTESIAN_POINT('Ctrl Pts',(-18.5220287095392,-21.058373026447,-2.10018006312557));
#77494=CARTESIAN_POINT('Ctrl Pts',(-18.5406629914278,-21.0601853086807,
-2.10129245268935));
#77495=CARTESIAN_POINT('Ctrl Pts',(-18.5522578105289,-21.061216508412,-2.10198106081862));
#77496=CARTESIAN_POINT('Ctrl Pts',(-18.6060541942796,-21.0655540526629,
-2.10516016387081));
#77497=CARTESIAN_POINT('Ctrl Pts',(-18.6483421141709,-21.0676899465985,
-2.10761379689482));
#77498=CARTESIAN_POINT('Ctrl Pts',(-18.7648645872267,-21.0700755020006,
-2.11427452492477));
#77499=CARTESIAN_POINT('Ctrl Pts',(-18.8390937832549,-21.0676921010481,
-2.11840428181186));
#77500=CARTESIAN_POINT('Ctrl Pts',(-19.0791534827002,-21.0473156275731,
-2.13162883027534));
#77501=CARTESIAN_POINT('Ctrl Pts',(-19.2429910353896,-21.0136485769753,
-2.14041564688287));
#77502=CARTESIAN_POINT('Ctrl Pts',(-19.434565167532,-20.9500330449553,-2.15196475350744));
#77503=CARTESIAN_POINT('Ctrl Pts',(-19.4676816584993,-20.9381114023114,
-2.15401157799856));
#77504=CARTESIAN_POINT('Ctrl Pts',(-19.5070465388779,-20.9228215601371,
-2.15652283454657));
#77505=CARTESIAN_POINT('Ctrl Pts',(-19.5135968095329,-20.9202396664534,
-2.15694334048251));
#77506=CARTESIAN_POINT('Ctrl Pts',(-19.5242950041681,-20.9159610204893,
-2.15763464107657));
#77507=CARTESIAN_POINT('Ctrl Pts',(-19.5284506947994,-20.914283663566,-2.15790429446698));
#77508=CARTESIAN_POINT('Ctrl Pts',(-19.5359015412223,-20.9112487384921,
-2.15838982847879));
#77509=CARTESIAN_POINT('Ctrl Pts',(-19.5391986201502,-20.9098960347546,
-2.15860541360415));
#77510=CARTESIAN_POINT('Ctrl Pts',(-19.54635659736,-20.906938168159,-2.15907505243277));
#77511=CARTESIAN_POINT('Ctrl Pts',(-19.5502161101035,-20.9053299115891,
-2.15932928787843));
#77512=CARTESIAN_POINT('Ctrl Pts',(-19.5609065938249,-20.9008379776625,
-2.16003625065996));
#77513=CARTESIAN_POINT('Ctrl Pts',(-19.5677271404579,-20.8979298624608,
-2.16049042168676));
#77514=CARTESIAN_POINT('Ctrl Pts',(-19.6072724394993,-20.8808226394272,
-2.16314130578718));
#77515=CARTESIAN_POINT('Ctrl Pts',(-19.6396473324771,-20.8658349168796,
-2.16538179422692));
#77516=CARTESIAN_POINT('Ctrl Pts',(-19.7424836811496,-20.8150340173786,
-2.17269150338552));
#77517=CARTESIAN_POINT('Ctrl Pts',(-19.8113211986012,-20.7760922234604,
-2.17788069750092));
#77518=CARTESIAN_POINT('Ctrl Pts',(-19.9507806423674,-20.6865468243716,
-2.18882077245553));
#77519=CARTESIAN_POINT('Ctrl Pts',(-20.0208012369451,-20.6352562117291,
-2.19456593442936));
#77520=CARTESIAN_POINT('Ctrl Pts',(-20.1722642798111,-20.5093190955114,
-2.20740013127517));
#77521=CARTESIAN_POINT('Ctrl Pts',(-20.2514210750559,-20.4322995660472,
-2.21440553909444));
#77522=CARTESIAN_POINT('Ctrl Pts',(-20.333587503665,-20.33879844327,-2.22200484823458));
#77523=CARTESIAN_POINT('Ctrl Pts',(-20.3428414896205,-20.3280520269145,
-2.22286616210404));
#77524=CARTESIAN_POINT('Ctrl Pts',(-20.3574188713835,-20.3107755946574,
-2.22423194628946));
#77525=CARTESIAN_POINT('Ctrl Pts',(-20.3628123594039,-20.3043055311788,
-2.22473928843057));
#77526=CARTESIAN_POINT('Ctrl Pts',(-20.3722685160257,-20.2928232145257,
-2.22563243727655));
#77527=CARTESIAN_POINT('Ctrl Pts',(-20.3763471297789,-20.2878242885755,
-2.22601888982665));
#77528=CARTESIAN_POINT('Ctrl Pts',(-20.3847473016138,-20.2774320457245,
-2.2268173959899));
#77529=CARTESIAN_POINT('Ctrl Pts',(-20.3890654343432,-20.2720360492813,
-2.22722930879292));
#77530=CARTESIAN_POINT('Ctrl Pts',(-20.4001056081468,-20.2581007634803,
-2.22828623475696));
#77531=CARTESIAN_POINT('Ctrl Pts',(-20.4067885119983,-20.2495306172316,
-2.22892968230987));
#77532=CARTESIAN_POINT('Ctrl Pts',(-20.4346053675792,-20.2132861943621,
-2.23162398089347));
#77533=CARTESIAN_POINT('Ctrl Pts',(-20.4551215893789,-20.1851432034442,
-2.23365053718074));
#77534=CARTESIAN_POINT('Ctrl Pts',(-20.5323186411735,-20.0735662598666,
-2.2414529178018));
#77535=CARTESIAN_POINT('Ctrl Pts',(-20.5837048545482,-19.9866283045965,
-2.2470334705779));
#77536=CARTESIAN_POINT('Ctrl Pts',(-20.663586701512,-19.8263570355579,-2.25680806958959));
#77537=CARTESIAN_POINT('Ctrl Pts',(-20.6945668143561,-19.7544852992699,
-2.26102665247313));
#77538=CARTESIAN_POINT('Ctrl Pts',(-20.7218604140742,-19.6800804036127,
-2.26535923033235));
#77539=CARTESIAN_POINT('Ctrl Pts',(-20.7222208667441,-19.6790955129461,
-2.26541657466571));
#77540=CARTESIAN_POINT('Ctrl Pts',(-20.7225805820961,-19.6781103693727,
-2.2654739284689));
#77541=CARTESIAN_POINT('Ctrl Pts',(-20.7225805826894,-19.6781103677477,
-2.04625070052543));
#77542=CARTESIAN_POINT('Ctrl Pts',(-20.7190678195543,-19.6877306856393,
-2.04566733720848));
#77543=CARTESIAN_POINT('Ctrl Pts',(-20.7154850976113,-19.6973259159891,
-2.04508122692791));
#77544=CARTESIAN_POINT('Ctrl Pts',(-20.7008062983039,-19.7357845066084,
-2.04271342574978));
#77545=CARTESIAN_POINT('Ctrl Pts',(-20.6891489348871,-19.7644269710652,
-2.04090765878723));
#77546=CARTESIAN_POINT('Ctrl Pts',(-20.6740381866449,-19.7993438756357,
-2.03864177403879));
#77547=CARTESIAN_POINT('Ctrl Pts',(-20.6711741826596,-19.8058711799589,
-2.03821537891728));
#77548=CARTESIAN_POINT('Ctrl Pts',(-20.6666170552106,-19.8161163151558,
-2.03754149041164));
#77549=CARTESIAN_POINT('Ctrl Pts',(-20.6649460105186,-19.8198439906011,
-2.03729532896267));
#77550=CARTESIAN_POINT('Ctrl Pts',(-20.6617920753461,-19.8268254112321,
-2.03683244207514));
#77551=CARTESIAN_POINT('Ctrl Pts',(-20.6603117271752,-19.8300802440396,
-2.03661587282193));
#77552=CARTESIAN_POINT('Ctrl Pts',(-20.6568999800089,-19.8375314827844,
-2.03611833908501));
#77553=CARTESIAN_POINT('Ctrl Pts',(-20.6549630922218,-19.8417253157622,
-2.03583703971688));
#77554=CARTESIAN_POINT('Ctrl Pts',(-20.6489187125119,-19.8547011241648,
-2.03496283317336));
#77555=CARTESIAN_POINT('Ctrl Pts',(-20.6447646756307,-19.863461102436,-2.0343671601292));
#77556=CARTESIAN_POINT('Ctrl Pts',(-20.5974979055914,-19.9613933702837,
-2.02764856428545));
#77557=CARTESIAN_POINT('Ctrl Pts',(-20.5482428284132,-20.0474532047992,
-2.02119626990881));
#77558=CARTESIAN_POINT('Ctrl Pts',(-20.3994673093771,-20.2696747704616,
-2.003579541899));
#77559=CARTESIAN_POINT('Ctrl Pts',(-20.2894008237162,-20.3979575619853,
-1.99239225570726));
#77560=CARTESIAN_POINT('Ctrl Pts',(-20.1424108759181,-20.532832482389,-1.97986538399193));
#77561=CARTESIAN_POINT('Ctrl Pts',(-20.1190797257721,-20.5533140988938,
-1.97793603921231));
#77562=CARTESIAN_POINT('Ctrl Pts',(-20.0837081766672,-20.5830138448141,
-1.97509657056978));
#77563=CARTESIAN_POINT('Ctrl Pts',(-20.07200638745,-20.5926270904666,-1.97417061497426));
#77564=CARTESIAN_POINT('Ctrl Pts',(-20.053101282801,-20.6078211857509,-1.97269574460927));
#77565=CARTESIAN_POINT('Ctrl Pts',(-20.0459635052767,-20.6134823978489,
-1.9721436156328));
#77566=CARTESIAN_POINT('Ctrl Pts',(-20.0322804493069,-20.6241917331012,
-1.97109407224112));
#77567=CARTESIAN_POINT('Ctrl Pts',(-20.0257417314927,-20.629247930227,-1.97059634135207));
#77568=CARTESIAN_POINT('Ctrl Pts',(-20.0142131900203,-20.6380552045011,
-1.96972538585768));
#77569=CARTESIAN_POINT('Ctrl Pts',(-20.0092361076183,-20.6418227231423,
-1.96935151439972));
#77570=CARTESIAN_POINT('Ctrl Pts',(-19.9993807200469,-20.6492146492863,
-1.96861535962426));
#77571=CARTESIAN_POINT('Ctrl Pts',(-19.9945033299632,-20.6528401714315,
-1.96825303480688));
#77572=CARTESIAN_POINT('Ctrl Pts',(-19.9828022176899,-20.6614600099083,
-1.96738851373889));
#77573=CARTESIAN_POINT('Ctrl Pts',(-19.9759640172694,-20.6664345678222,
-1.96688708763631));
#77574=CARTESIAN_POINT('Ctrl Pts',(-19.951156598313,-20.6842548049735,-1.96508152989753));
#77575=CARTESIAN_POINT('Ctrl Pts',(-19.9330160197317,-20.6968603189806,
-1.96378661516836));
#77576=CARTESIAN_POINT('Ctrl Pts',(-19.7605316039865,-20.8127557130371,
-1.95170046419682));
#77577=CARTESIAN_POINT('Ctrl Pts',(-19.5934291011689,-20.8955963013441,
-1.94176724924772));
#77578=CARTESIAN_POINT('Ctrl Pts',(-19.3418755601045,-20.9814300818394,
-1.92727730385095));
#77579=CARTESIAN_POINT('Ctrl Pts',(-19.2647017150212,-21.0029638809598,
-1.92287411277622));
#77580=CARTESIAN_POINT('Ctrl Pts',(-19.1513240644229,-21.0277712470727,
-1.91623522899354));
#77581=CARTESIAN_POINT('Ctrl Pts',(-19.1159589849224,-21.0345687577443,
-1.91414068824534));
#77582=CARTESIAN_POINT('Ctrl Pts',(-19.0730758941525,-21.0416823356312,
-1.91155379071));
#77583=CARTESIAN_POINT('Ctrl Pts',(-19.0657052693835,-21.0428649732448,
-1.91110749168472));
#77584=CARTESIAN_POINT('Ctrl Pts',(-19.0542187151086,-21.0446457588916,
-1.91040915479717));
#77585=CARTESIAN_POINT('Ctrl Pts',(-19.0501069330924,-21.0452708147491,
-1.9101586142393));
#77586=CARTESIAN_POINT('Ctrl Pts',(-19.0424663468632,-21.0464092792429,
-1.90969197025716));
#77587=CARTESIAN_POINT('Ctrl Pts',(-19.0389380777652,-21.046925889918,-1.90947605030773));
#77588=CARTESIAN_POINT('Ctrl Pts',(-19.0309434826086,-21.0480758376547,
-1.90898582900953));
#77589=CARTESIAN_POINT('Ctrl Pts',(-19.026476449865,-21.0487038118119,-1.90871122998497));
#77590=CARTESIAN_POINT('Ctrl Pts',(-19.0149365151976,-21.0502884968433,
-1.9080001362419));
#77591=CARTESIAN_POINT('Ctrl Pts',(-19.0078607872201,-21.0512237154404,
-1.90756247410033));
#77592=CARTESIAN_POINT('Ctrl Pts',(-18.9643580473622,-21.056749908699,-1.90486206382203));
#77593=CARTESIAN_POINT('Ctrl Pts',(-18.9278237679634,-21.0604280827711,
-1.90255300475009));
#77594=CARTESIAN_POINT('Ctrl Pts',(-18.7213462194097,-21.075804206797,-1.88933906323761));
#77595=CARTESIAN_POINT('Ctrl Pts',(-18.5505732804184,-21.0679069289307,
-1.87784579016391));
#77596=CARTESIAN_POINT('Ctrl Pts',(-18.288426158339,-21.0237796023901,-1.86056924249069));
#77597=CARTESIAN_POINT('Ctrl Pts',(-18.1954346426859,-21.00157517292,-1.85450219355194));
#77598=CARTESIAN_POINT('Ctrl Pts',(-18.0838141290484,-20.966796629113,-1.84732064884633));
#77599=CARTESIAN_POINT('Ctrl Pts',(-18.0634764335022,-20.9601198477793,
-1.84601599339661));
#77600=CARTESIAN_POINT('Ctrl Pts',(-18.0347242032187,-20.9501950792171,
-1.84417645125597));
#77601=CARTESIAN_POINT('Ctrl Pts',(-18.0262242790272,-20.94720017725,-1.84363324546491));
#77602=CARTESIAN_POINT('Ctrl Pts',(-18.0116017707027,-20.941942812525,-1.84269974461762));
#77603=CARTESIAN_POINT('Ctrl Pts',(-18.0054700997176,-20.9397061615559,
-1.84230859794233));
#77604=CARTESIAN_POINT('Ctrl Pts',(-17.9937551270939,-20.935371397761,-1.84156182277498));
#77605=CARTESIAN_POINT('Ctrl Pts',(-17.9881701658856,-20.9332779797359,
-1.84120604210323));
#77606=CARTESIAN_POINT('Ctrl Pts',(-17.9736824205417,-20.9277775794377,
-1.84028369350109));
#77607=CARTESIAN_POINT('Ctrl Pts',(-17.9647936043243,-20.9243339956537,
-1.83971835628536));
#77608=CARTESIAN_POINT('Ctrl Pts',(-17.9346247699119,-20.9124114260076,
-1.83780125513713));
#77609=CARTESIAN_POINT('Ctrl Pts',(-17.9134587713652,-20.9036469634844,
-1.8364591005122));
#77610=CARTESIAN_POINT('Ctrl Pts',(-17.730397719994,-20.8243399290242,-1.82486537947046));
#77611=CARTESIAN_POINT('Ctrl Pts',(-17.577778751225,-20.734142928077,-1.8153758609545));
#77612=CARTESIAN_POINT('Ctrl Pts',(-17.3699361942469,-20.5732507793918,
-1.80107191152797));
#77613=CARTESIAN_POINT('Ctrl Pts',(-17.3050449697912,-20.5163558826288,
-1.7963489923218));
#77614=CARTESIAN_POINT('Ctrl Pts',(-17.2170838455513,-20.4291831592641,
-1.78927699853988));
#77615=CARTESIAN_POINT('Ctrl Pts',(-17.1910715232213,-20.4019917336887,
-1.7870910913466));
#77616=CARTESIAN_POINT('Ctrl Pts',(-17.1607205265127,-20.3685231584339,
-1.78440287333128));
#77617=CARTESIAN_POINT('Ctrl Pts',(-17.1556718303541,-20.3628955826249,
-1.78395093746037));
#77618=CARTESIAN_POINT('Ctrl Pts',(-17.1478789475879,-20.3541150017325,
-1.78324568424477));
#77619=CARTESIAN_POINT('Ctrl Pts',(-17.1451137141005,-20.3509806434598,
-1.78299391256094));
#77620=CARTESIAN_POINT('Ctrl Pts',(-17.1400079158395,-20.3451586189318,
-1.78252616633747));
#77621=CARTESIAN_POINT('Ctrl Pts',(-17.1376648487835,-20.342473223862,-1.78231038280618));
#77622=CARTESIAN_POINT('Ctrl Pts',(-17.1323896226924,-20.3363963661908,
-1.78182200170695));
#77623=CARTESIAN_POINT('Ctrl Pts',(-17.1294614661708,-20.3330015177484,
-1.78154911600803));
#77624=CARTESIAN_POINT('Ctrl Pts',(-17.1208694787161,-20.3229759179436,
-1.78074315403428));
#77625=CARTESIAN_POINT('Ctrl Pts',(-17.115235889878,-20.3163195359043,-1.78020794081838));
#77626=CARTESIAN_POINT('Ctrl Pts',(-17.0754251888519,-20.2686873928663,
-1.77637848201504));
#77627=CARTESIAN_POINT('Ctrl Pts',(-17.0427697643961,-20.226470614844,-1.77298712418771));
#77628=CARTESIAN_POINT('Ctrl Pts',(-17.0014762191369,-20.168701394637,-1.76839776225945));
#77629=CARTESIAN_POINT('Ctrl Pts',(-16.9913860734998,-20.1542053126184,
-1.76725022502634));
#77630=CARTESIAN_POINT('Ctrl Pts',(-16.9543026867097,-20.0994812912088,
-1.76293769807455));
#77631=CARTESIAN_POINT('Ctrl Pts',(-16.9285119216045,-20.058457591769,-1.75974409731762));
#77632=CARTESIAN_POINT('Ctrl Pts',(-16.849146026128,-19.9220407382868,-1.74931865084814));
#77633=CARTESIAN_POINT('Ctrl Pts',(-16.8015463320435,-19.8233666414338,
-1.742085863055));
#77634=CARTESIAN_POINT('Ctrl Pts',(-16.7417568175448,-19.6701171705583,
-1.73151222865472));
#77635=CARTESIAN_POINT('Ctrl Pts',(-16.7237400582286,-19.6180187356863,
-1.72802300287674));
#77636=CARTESIAN_POINT('Ctrl Pts',(-16.6978381781391,-19.5324401562204,
-1.72246531640385));
#77637=CARTESIAN_POINT('Ctrl Pts',(-16.6886998391823,-19.4993693526762,
-1.72035841402675));
#77638=CARTESIAN_POINT('Ctrl Pts',(-16.6777441292952,-19.4556046220498,
-1.71762185256941));
#77639=CARTESIAN_POINT('Ctrl Pts',(-16.6751997329276,-19.4450996737436,
-1.71696885089705));
#77640=CARTESIAN_POINT('Ctrl Pts',(-16.6711634629899,-19.4278592259875,
-1.71590335916471));
#77641=CARTESIAN_POINT('Ctrl Pts',(-16.6696238845251,-19.4211352011839,
-1.7154893396334));
#77642=CARTESIAN_POINT('Ctrl Pts',(-16.6667069027187,-19.4081029904322,
-1.71468983673421));
#77643=CARTESIAN_POINT('Ctrl Pts',(-16.6653254418001,-19.4017957999248,
-1.71430422701255));
#77644=CARTESIAN_POINT('Ctrl Pts',(-16.6622017609047,-19.3872155026155,
-1.7134158266876));
#77645=CARTESIAN_POINT('Ctrl Pts',(-16.6604801942873,-19.378938046695,-1.71291370211267));
#77646=CARTESIAN_POINT('Ctrl Pts',(-16.6559824447547,-19.3566433286995,
-1.71156713494216));
#77647=CARTESIAN_POINT('Ctrl Pts',(-16.6532984879279,-19.3426077520206,
-1.710725633561));
#77648=CARTESIAN_POINT('Ctrl Pts',(-16.6299803466818,-19.2135999198293,
-1.70304546140456));
#77649=CARTESIAN_POINT('Ctrl Pts',(-16.6187512461435,-19.0971247379113,
-1.69652331624241));
#77650=CARTESIAN_POINT('Ctrl Pts',(-16.6150141574696,-18.8176357478624,
-1.68122134773218));
#77651=CARTESIAN_POINT('Ctrl Pts',(-16.6315967213824,-18.6552789540971,
-1.67262441655658));
#77652=CARTESIAN_POINT('Ctrl Pts',(-16.6736069919899,-18.4646285363578,
-1.6614158197078));
#77653=CARTESIAN_POINT('Ctrl Pts',(-16.6813503331717,-18.4329822994738,
-1.65951585324633));
#77654=CARTESIAN_POINT('Ctrl Pts',(-16.6917038813867,-18.3945342674246,
-1.6571450963628));
#77655=CARTESIAN_POINT('Ctrl Pts',(-16.693623420371,-18.3875490376032,-1.65671183579415));
#77656=CARTESIAN_POINT('Ctrl Pts',(-16.6966883047469,-18.376615820509,-1.65602951244593));
#77657=CARTESIAN_POINT('Ctrl Pts',(-16.697809383091,-18.3726610072034,-1.65578183773681));
#77658=CARTESIAN_POINT('Ctrl Pts',(-16.6999260702594,-18.3652760396696,
-1.6553176910471));
#77659=CARTESIAN_POINT('Ctrl Pts',(-16.7009188438121,-18.3618451313637,
-1.6551013848204));
#77660=CARTESIAN_POINT('Ctrl Pts',(-16.7032044325518,-18.3540206205047,
-1.65460654986977));
#77661=CARTESIAN_POINT('Ctrl Pts',(-16.7045028212763,-18.3496287061034,
-1.65432769981613));
#77662=CARTESIAN_POINT('Ctrl Pts',(-16.7085359774964,-18.3361472639435,
-1.65346843807196));
#77663=CARTESIAN_POINT('Ctrl Pts',(-16.7113175908226,-18.3270720338653,
-1.65288539238236));
#77664=CARTESIAN_POINT('Ctrl Pts',(-16.7367707030987,-18.2459797455049,
-1.64763601863469));
#77665=CARTESIAN_POINT('Ctrl Pts',(-16.7632164951043,-18.1752121733009,
-1.64277665110504));
#77666=CARTESIAN_POINT('Ctrl Pts',(-16.8475005998302,-17.9818711473493,
-1.62898457159768));
#77667=CARTESIAN_POINT('Ctrl Pts',(-16.9134127660971,-17.863195252135,-1.61993219658966));
#77668=CARTESIAN_POINT('Ctrl Pts',(-17.041206518941,-17.6775479604834,-1.6053260997555));
#77669=CARTESIAN_POINT('Ctrl Pts',(-17.0968763104419,-17.6067835132174,
-1.59962665350095));
#77670=CARTESIAN_POINT('Ctrl Pts',(-17.170716119228,-17.5243227584686,-1.59283208250353));
#77671=CARTESIAN_POINT('Ctrl Pts',(-17.1847724627518,-17.5090818167031,
-1.59156897800392));
#77672=CARTESIAN_POINT('Ctrl Pts',(-17.2051781508662,-17.4875984456937,
-1.58977741907538));
#77673=CARTESIAN_POINT('Ctrl Pts',(-17.2113461565476,-17.4811861316128,
-1.58924122423206));
#77674=CARTESIAN_POINT('Ctrl Pts',(-17.2220942905375,-17.4701523507733,
-1.58831597872501));
#77675=CARTESIAN_POINT('Ctrl Pts',(-17.2266556019151,-17.4655127996336,
-1.58792611600589));
#77676=CARTESIAN_POINT('Ctrl Pts',(-17.2354566220657,-17.4566429815126,
-1.58717918400606));
#77677=CARTESIAN_POINT('Ctrl Pts',(-17.2396930294272,-17.4524095402002,
-1.58682197507435));
#77678=CARTESIAN_POINT('Ctrl Pts',(-17.2508148454768,-17.4413894403611,
-1.58589021910236));
#77679=CARTESIAN_POINT('Ctrl Pts',(-17.2577289288232,-17.434631819693,-1.58531695388658));
#77680=CARTESIAN_POINT('Ctrl Pts',(-17.2817684682588,-17.4114561361086,
-1.58334401763752));
#77681=CARTESIAN_POINT('Ctrl Pts',(-17.2991238359299,-17.3952783553431,
-1.58195474199971));
#77682=CARTESIAN_POINT('Ctrl Pts',(-17.4372484007768,-17.2707986906363,
-1.57115794072198));
#77683=CARTESIAN_POINT('Ctrl Pts',(-17.5698311025968,-17.1764098680476,
-1.56237647059935));
#77684=CARTESIAN_POINT('Ctrl Pts',(-17.8260773644939,-17.0351372980038,
-1.54648015492268));
#77685=CARTESIAN_POINT('Ctrl Pts',(-17.9458033605028,-16.9828828586032,
-1.53938988112134));
#77686=CARTESIAN_POINT('Ctrl Pts',(-18.0808437687644,-16.9382429733636,
-1.53099659419024));
#77687=CARTESIAN_POINT('Ctrl Pts',(-18.0921660077211,-16.9346057558173,
-1.53028986634222));
#77688=CARTESIAN_POINT('Ctrl Pts',(-18.1083101308925,-16.9295691884824,
-1.52927710045089));
#77689=CARTESIAN_POINT('Ctrl Pts',(-18.1131075134792,-16.9280912276785,
-1.528975515019));
#77690=CARTESIAN_POINT('Ctrl Pts',(-18.1213859413958,-16.925573042289,-1.52845393404589));
#77691=CARTESIAN_POINT('Ctrl Pts',(-18.1248645276573,-16.9245246793309,
-1.52823441316264));
#77692=CARTESIAN_POINT('Ctrl Pts',(-18.1316161213705,-16.9225088541225,
-1.52780763364235));
#77693=CARTESIAN_POINT('Ctrl Pts',(-18.1348887764096,-16.9215403501145,
-1.52760044324629));
#77694=CARTESIAN_POINT('Ctrl Pts',(-18.1437280857569,-16.9189476905458,
-1.52703999354796));
#77695=CARTESIAN_POINT('Ctrl Pts',(-18.1492990466822,-16.9173385001205,
-1.52668587665264));
#77696=CARTESIAN_POINT('Ctrl Pts',(-18.1700200047351,-16.9114453104256,
-1.52536561859706));
#77697=CARTESIAN_POINT('Ctrl Pts',(-18.1852106047553,-16.9073075922571,
-1.52439152156402));
#77698=CARTESIAN_POINT('Ctrl Pts',(-18.3278408526358,-16.870160864034,-1.51519649801879));
#77699=CARTESIAN_POINT('Ctrl Pts',(-18.4580418341895,-16.8489402244129,
-1.50645731733271));
#77700=CARTESIAN_POINT('Ctrl Pts',(-18.7482991390137,-16.8290619672997,
-1.487239119146));
#77701=CARTESIAN_POINT('Ctrl Pts',(-18.9079913130624,-16.8361513367251,
-1.47686732231346));
#77702=CARTESIAN_POINT('Ctrl Pts',(-19.0864171272193,-16.8644310703918,
-1.46577186590442));
#77703=CARTESIAN_POINT('Ctrl Pts',(-19.1073845944292,-16.8680792088082,
-1.46447482370769));
#77704=CARTESIAN_POINT('Ctrl Pts',(-19.1371281389595,-16.8737176447483,
-1.46264404197272));
#77705=CARTESIAN_POINT('Ctrl Pts',(-19.1459515159648,-16.8754485807078,
-1.46210209142977));
#77706=CARTESIAN_POINT('Ctrl Pts',(-19.1611568616866,-16.8785322358493,
-1.46117005519189));
#77707=CARTESIAN_POINT('Ctrl Pts',(-19.1675440460578,-16.8798583264978,
-1.46077912511099));
#77708=CARTESIAN_POINT('Ctrl Pts',(-19.179763779525,-16.8824543295307,-1.46003229214783));
#77709=CARTESIAN_POINT('Ctrl Pts',(-19.185597277295,-16.8837194267803,-1.45967623934523));
#77710=CARTESIAN_POINT('Ctrl Pts',(-19.2007565986014,-16.8870741869795,
-1.45875216575367));
#77711=CARTESIAN_POINT('Ctrl Pts',(-19.2100738278235,-16.8892023728368,
-1.45818538481364));
#77712=CARTESIAN_POINT('Ctrl Pts',(-19.2418171654502,-16.8966795253776,
-1.45625815048359));
#77713=CARTESIAN_POINT('Ctrl Pts',(-19.2641706545985,-16.9023318157934,
-1.45490744634196));
#77714=CARTESIAN_POINT('Ctrl Pts',(-19.4549976985346,-16.953915070331,-1.44342150463895));
#77715=CARTESIAN_POINT('Ctrl Pts',(-19.6172807621166,-17.0201607465475,
-1.43402853690495));
#77716=CARTESIAN_POINT('Ctrl Pts',(-19.8460091767101,-17.1484479468382,
-1.41976125585502));
#77717=CARTESIAN_POINT('Ctrl Pts',(-19.9196806860506,-17.1960036168401,
-1.41496687862995));
#77718=CARTESIAN_POINT('Ctrl Pts',(-20.0207562178372,-17.2705156446807,
-1.40779853363121));
#77719=CARTESIAN_POINT('Ctrl Pts',(-20.050710172864,-17.2938669781061,-1.40559284897915));
#77720=CARTESIAN_POINT('Ctrl Pts',(-20.0858688090117,-17.3228292943661,
-1.40288270525609));
#77721=CARTESIAN_POINT('Ctrl Pts',(-20.0916937757686,-17.3276804279405,
-1.40242958083281));
#77722=CARTESIAN_POINT('Ctrl Pts',(-20.1006932809881,-17.3352576013287,
-1.40172286696889));
#77723=CARTESIAN_POINT('Ctrl Pts',(-20.1038860708932,-17.3379620016751,
-1.40147083342189));
#77724=CARTESIAN_POINT('Ctrl Pts',(-20.1097830114752,-17.342987009666,-1.40100286219437));
#77725=CARTESIAN_POINT('Ctrl Pts',(-20.1124893284976,-17.3453049858886,
-1.40078711718446));
#77726=CARTESIAN_POINT('Ctrl Pts',(-20.118582736565,-17.3505507532902,-1.40029915277496));
#77727=CARTESIAN_POINT('Ctrl Pts',(-20.1219663794784,-17.3534824452741,
-1.4000266473414));
#77728=CARTESIAN_POINT('Ctrl Pts',(-20.1318927169114,-17.3621382059273,
-1.3992227406268));
#77729=CARTESIAN_POINT('Ctrl Pts',(-20.138409390065,-17.367891786714,-1.39868921784563));
#77730=CARTESIAN_POINT('Ctrl Pts',(-20.1842716029898,-17.4088890282016,
-1.39489468584104));
#77731=CARTESIAN_POINT('Ctrl Pts',(-20.2223180985812,-17.4455513876767,
-1.39153847472474));
#77732=CARTESIAN_POINT('Ctrl Pts',(-20.2724921201232,-17.4976574855266,
-1.38686505684447));
#77733=CARTESIAN_POINT('Ctrl Pts',(-20.2858384035778,-17.5119070552806,
-1.38559624901655));
#77734=CARTESIAN_POINT('Ctrl Pts',(-20.397595909335,-17.6345861820864,-1.37476371728557));
#77735=CARTESIAN_POINT('Ctrl Pts',(-20.4847190246882,-17.7527841633212,
-1.3649584311791));
#77736=CARTESIAN_POINT('Ctrl Pts',(-20.5902290778054,-17.9322388444991,
-1.35150933953882));
#77737=CARTESIAN_POINT('Ctrl Pts',(-20.6191743280918,-17.9867963515892,
-1.34758323029188));
#77738=CARTESIAN_POINT('Ctrl Pts',(-20.6616864855659,-18.0761579328442,
-1.34141723280114));
#77739=CARTESIAN_POINT('Ctrl Pts',(-20.6767885701733,-18.1101880490366,
-1.3391275721287));
#77740=CARTESIAN_POINT('Ctrl Pts',(-20.6952311453368,-18.1548894204109,
-1.33619300060901));
#77741=CARTESIAN_POINT('Ctrl Pts',(-20.6993949332349,-18.1652118167138,
-1.33552031141605));
#77742=CARTESIAN_POINT('Ctrl Pts',(-20.7060328960241,-18.1820494725962,
-1.33443094956885));
#77743=CARTESIAN_POINT('Ctrl Pts',(-20.7085566090558,-18.1885448558746,
-1.3340126126734));
#77744=CARTESIAN_POINT('Ctrl Pts',(-20.7133473748445,-18.2010577141666,
-1.33321032421712));
#77745=CARTESIAN_POINT('Ctrl Pts',(-20.7156191687908,-18.207073279949,-1.33282621705269));
#77746=CARTESIAN_POINT('Ctrl Pts',(-20.7207568509151,-18.2208673638336,
-1.33194903142352));
#77747=CARTESIAN_POINT('Ctrl Pts',(-20.7236045418523,-18.2286525825372,
-1.33145656532494));
#77748=CARTESIAN_POINT('Ctrl Pts',(-20.7310458567812,-18.2493726096214,
-1.33015267371095));
#77749=CARTESIAN_POINT('Ctrl Pts',(-20.7355595833636,-18.262335841672,-1.32934390222874));
#77750=CARTESIAN_POINT('Ctrl Pts',(-20.768858789551,-18.3610511026393,-1.32323614162636));
#77751=CARTESIAN_POINT('Ctrl Pts',(-20.7922497677207,-18.4485303721536,
-1.31812045243364));
#77752=CARTESIAN_POINT('Ctrl Pts',(-20.8373639019983,-18.6743412751769,
-1.30537420899799));
#77753=CARTESIAN_POINT('Ctrl Pts',(-20.8511051846576,-18.813805234618,-1.29793914602196));
#77754=CARTESIAN_POINT('Ctrl Pts',(-20.850984040619,-18.9738904697264,-1.28909422412968));
#77755=CARTESIAN_POINT('Ctrl Pts',(-20.8506770343583,-18.9941772551681,
-1.28796714642275));
#77756=CARTESIAN_POINT('Ctrl Pts',(-20.8483264232153,-19.0738184747613,
-1.2835078783363));
#77757=CARTESIAN_POINT('Ctrl Pts',(-20.8440773310445,-19.1330752901755,
-1.28011463463512));
#77758=CARTESIAN_POINT('Ctrl Pts',(-20.836329718907,-19.2009553113883,-1.27606208409883));
#77759=CARTESIAN_POINT('Ctrl Pts',(-20.8352591869441,-19.209834863776,-1.27552867654599));
#77760=CARTESIAN_POINT('Ctrl Pts',(-20.8335616366235,-19.2232018844552,
-1.27472039173358));
#77761=CARTESIAN_POINT('Ctrl Pts',(-20.8329764090901,-19.2276946885955,
-1.27444781320648));
#77762=CARTESIAN_POINT('Ctrl Pts',(-20.831904658458,-19.2357212866073,-1.2739591658741));
#77763=CARTESIAN_POINT('Ctrl Pts',(-20.8314236225286,-19.2392557603419,
-1.27374340933918));
#77764=CARTESIAN_POINT('Ctrl Pts',(-20.830364447558,-19.2468936671231,-1.27327589048336));
#77765=CARTESIAN_POINT('Ctrl Pts',(-20.8297832007567,-19.2509965662683,
-1.27302395992035));
#77766=CARTESIAN_POINT('Ctrl Pts',(-20.8281309522132,-19.2624178821841,
-1.27232050370401));
#77767=CARTESIAN_POINT('Ctrl Pts',(-20.8270336493153,-19.2697323491824,
-1.2718675311357));
#77768=CARTESIAN_POINT('Ctrl Pts',(-20.8205389602655,-19.3115308797211,
-1.26926550463275));
#77769=CARTESIAN_POINT('Ctrl Pts',(-20.8143280491217,-19.3458809039005,
-1.26707454839359));
#77770=CARTESIAN_POINT('Ctrl Pts',(-20.791895818292,-19.4545296439919,-1.26000957896572));
#77771=CARTESIAN_POINT('Ctrl Pts',(-20.7725200301541,-19.5281126177893,
-1.25502394121134));
#77772=CARTESIAN_POINT('Ctrl Pts',(-20.7408447920318,-19.6265459931844,
-1.24820178648662));
#77773=CARTESIAN_POINT('Ctrl Pts',(-20.7319594894793,-19.6524245799638,
-1.2463931639016));
#77774=CARTESIAN_POINT('Ctrl Pts',(-20.7225806439552,-19.6781101999604,
-1.24458624895942));
#77775=CARTESIAN_POINT('Origin',(-18.734,-18.952,0.));
#77776=CARTESIAN_POINT('',(-20.7225805821191,-19.6781103693095,-0.444429623604461));
#77777=CARTESIAN_POINT('',(-20.7225805821191,-19.6781103693095,-0.666446455478431));
#77778=CARTESIAN_POINT('',(-20.7225805821191,-19.6781103693095,0.));
#77779=CARTESIAN_POINT('',(-17.1140743056112,-17.5890877707427,0.));
#77780=CARTESIAN_POINT('Ctrl Pts',(-20.7225805821191,-19.6781103693095,
-0.444429623604461));
#77781=CARTESIAN_POINT('Ctrl Pts',(-20.6978890887291,-19.7457323540302,
-0.440115259735745));
#77782=CARTESIAN_POINT('Ctrl Pts',(-20.66973990691,-19.8121053494161,-0.435800895867028));
#77783=CARTESIAN_POINT('Ctrl Pts',(-20.6382937703335,-19.8768536296458,
-0.431486531998312));
#77784=CARTESIAN_POINT('Ctrl Pts',(-20.6068209446005,-19.94165686343,-0.427168506416429));
#77785=CARTESIAN_POINT('Ctrl Pts',(-20.5720457909348,-20.00483217924,-0.422850480834545));
#77786=CARTESIAN_POINT('Ctrl Pts',(-20.5341758415686,-20.0660269024726,
-0.418532455252662));
#77787=CARTESIAN_POINT('Ctrl Pts',(-20.4962904232958,-20.127246622186,-0.41421266586766));
#77788=CARTESIAN_POINT('Ctrl Pts',(-20.4553079752336,-20.1864837294646,
-0.409892876482659));
#77789=CARTESIAN_POINT('Ctrl Pts',(-20.4114787744278,-20.2434154874959,
-0.405573087097658));
#77790=CARTESIAN_POINT('Ctrl Pts',(-20.3675728005617,-20.3004469695743,
-0.401245730988999));
#77791=CARTESIAN_POINT('Ctrl Pts',(-20.3208104379345,-20.3551646589689,
-0.39691837488034));
#77792=CARTESIAN_POINT('Ctrl Pts',(-20.271481107869,-20.4072803313953,-0.392591018771681));
#77793=CARTESIAN_POINT('Ctrl Pts',(-20.2294415884618,-20.4516944318802,
-0.388903152529222));
#77794=CARTESIAN_POINT('Ctrl Pts',(-20.1855384971826,-20.4942192435085,
-0.385215286286762));
#77795=CARTESIAN_POINT('Ctrl Pts',(-20.1399695482849,-20.534699791273,-0.381527420044303));
#77796=CARTESIAN_POINT('Ctrl Pts',(-20.0856805306588,-20.5829266919205,
-0.377133844149252));
#77797=CARTESIAN_POINT('Ctrl Pts',(-20.0288042210985,-20.628448612849,-0.372740268254202));
#77798=CARTESIAN_POINT('Ctrl Pts',(-19.9696409341316,-20.6709765797993,
-0.368346692359152));
#77799=CARTESIAN_POINT('Ctrl Pts',(-19.9105639455,-20.7134425134695,-0.363959525139234));
#77800=CARTESIAN_POINT('Ctrl Pts',(-19.8492069897094,-20.7529228848838,
-0.359572357919316));
#77801=CARTESIAN_POINT('Ctrl Pts',(-19.7859047362903,-20.7891677728967,
-0.355185190699398));
#77802=CARTESIAN_POINT('Ctrl Pts',(-19.722674949545,-20.8253711687613,-0.350803045787515));
#77803=CARTESIAN_POINT('Ctrl Pts',(-19.65750470457,-20.8583462016274,-0.346420900875633));
#77804=CARTESIAN_POINT('Ctrl Pts',(-19.5907576513137,-20.8878861864571,
-0.34203875596375));
#77805=CARTESIAN_POINT('Ctrl Pts',(-19.5240517390545,-20.9174079636751,
-0.337659312082134));
#77806=CARTESIAN_POINT('Ctrl Pts',(-19.4557713858207,-20.9434987000513,
-0.333279868200517));
#77807=CARTESIAN_POINT('Ctrl Pts',(-19.38630358708,-20.9659982696821,-0.328900424318901));
#77808=CARTESIAN_POINT('Ctrl Pts',(-19.3168558633838,-20.9884913373096,
-0.324522246024118));
#77809=CARTESIAN_POINT('Ctrl Pts',(-19.2462218327665,-21.0073951506619,
-0.320144067729335));
#77810=CARTESIAN_POINT('Ctrl Pts',(-19.1748055877232,-21.0225988104488,
-0.315765889434552));
#77811=CARTESIAN_POINT('Ctrl Pts',(-19.1033866007398,-21.0378030539618,
-0.311387543044916));
#77812=CARTESIAN_POINT('Ctrl Pts',(-19.0311858104649,-21.0493067636484,
-0.30700919665528));
#77813=CARTESIAN_POINT('Ctrl Pts',(-18.9586178566871,-21.0570500750475,
-0.302630850265644));
#77814=CARTESIAN_POINT('Ctrl Pts',(-18.8859739522816,-21.0648014907037,
-0.298247921437905));
#77815=CARTESIAN_POINT('Ctrl Pts',(-18.8129625963386,-21.0687845992062,
-0.293864992610166));
#77816=CARTESIAN_POINT('Ctrl Pts',(-18.7400030989877,-21.0689914885995,
-0.289482063782427));
#77817=CARTESIAN_POINT('Ctrl Pts',(-18.6670032476661,-21.0691984924235,
-0.285096710752382));
#77818=CARTESIAN_POINT('Ctrl Pts',(-18.5940557926886,-21.0656251419751,
-0.280711357722337));
#77819=CARTESIAN_POINT('Ctrl Pts',(-18.5215768813659,-21.0583156028169,
-0.276326004692292));
#77820=CARTESIAN_POINT('Ctrl Pts',(-18.4489698822544,-21.0509931459328,
-0.271932901681429));
#77821=CARTESIAN_POINT('Ctrl Pts',(-18.3768335560974,-21.039921387774,-0.267539798670566));
#77822=CARTESIAN_POINT('Ctrl Pts',(-18.3055752234051,-21.0251958930115,
-0.263146695659703));
#77823=CARTESIAN_POINT('Ctrl Pts',(-18.2580216757331,-21.0153689788707,
-0.260215001560758));
#77824=CARTESIAN_POINT('Ctrl Pts',(-18.210858896598,-21.0039159582902,-0.257283307461813));
#77825=CARTESIAN_POINT('Ctrl Pts',(-18.164203666426,-20.9908774210937,-0.254351613362869));
#77826=CARTESIAN_POINT('Ctrl Pts',(-18.0951064200439,-20.9715671098208,
-0.250009720959284));
#77827=CARTESIAN_POINT('Ctrl Pts',(-18.0268407868783,-20.9486978630522,
-0.245667828555699));
#77828=CARTESIAN_POINT('Ctrl Pts',(-17.9598054524231,-20.922358292926,-0.241325936152114));
#77829=CARTESIAN_POINT('Ctrl Pts',(-17.8928710627946,-20.8960583861112,
-0.236990581965715));
#77830=CARTESIAN_POINT('Ctrl Pts',(-17.8271637514137,-20.8662987014601,
-0.232655227779317));
#77831=CARTESIAN_POINT('Ctrl Pts',(-17.763068724128,-20.8332180781434,-0.228319873592918));
#77832=CARTESIAN_POINT('Ctrl Pts',(-17.699047363678,-20.8001754756366,-0.223989502192827));
#77833=CARTESIAN_POINT('Ctrl Pts',(-17.6366350451716,-20.7638197356247,
-0.219659130792735));
#77834=CARTESIAN_POINT('Ctrl Pts',(-17.5761969042586,-20.7243377193672,
-0.215328759392644));
#77835=CARTESIAN_POINT('Ctrl Pts',(-17.5157959073165,-20.6848799679007,
-0.211001049344912));
#77836=CARTESIAN_POINT('Ctrl Pts',(-17.457367094634,-20.6423000184136,-0.206673339297181));
#77837=CARTESIAN_POINT('Ctrl Pts',(-17.4012494835622,-20.5968297969501,
-0.202345629249449));
#77838=CARTESIAN_POINT('Ctrl Pts',(-17.3451469193491,-20.5513717674523,
-0.198019079593976));
#77839=CARTESIAN_POINT('Ctrl Pts',(-17.2913547105839,-20.5030253137849,
-0.193692529938503));
#77840=CARTESIAN_POINT('Ctrl Pts',(-17.2401799611388,-20.4520635624855,
-0.18936598028303));
#77841=CARTESIAN_POINT('Ctrl Pts',(-17.1890012037485,-20.4010978199226,
-0.185039091777358));
#77842=CARTESIAN_POINT('Ctrl Pts',(-17.1404406606225,-20.3475167229364,
-0.180712203271685));
#77843=CARTESIAN_POINT('Ctrl Pts',(-17.0947683110377,-20.2916299749938,
-0.176385314766013));
#77844=CARTESIAN_POINT('Ctrl Pts',(-17.0490411502534,-20.2356761575941,
-0.172053233579186));
#77845=CARTESIAN_POINT('Ctrl Pts',(-17.0062094147358,-20.1774115489121,
-0.167721152392358));
#77846=CARTESIAN_POINT('Ctrl Pts',(-16.9665019464716,-20.1171779395326,
-0.16338907120553));
#77847=CARTESIAN_POINT('Ctrl Pts',(-16.9267699714228,-20.0569071549778,
-0.159054316330717));
#77848=CARTESIAN_POINT('Ctrl Pts',(-16.8901663478009,-19.9946653786934,
-0.154719561455904));
#77849=CARTESIAN_POINT('Ctrl Pts',(-16.8568742859376,-19.9308197247736,
-0.150384806581091));
#77850=CARTESIAN_POINT('Ctrl Pts',(-16.8235151748393,-19.8668454875814,
-0.146041321637236));
#77851=CARTESIAN_POINT('Ctrl Pts',(-16.793481145719,-19.8012613727176,-0.141697836693382));
#77852=CARTESIAN_POINT('Ctrl Pts',(-16.7669073048299,-19.7344546815047,
-0.137354351749528));
#77853=CARTESIAN_POINT('Ctrl Pts',(-16.7461495461317,-19.6822696330047,
-0.133961503393496));
#77854=CARTESIAN_POINT('Ctrl Pts',(-16.7275021235515,-19.6293390357121,
-0.130568655037465));
#77855=CARTESIAN_POINT('Ctrl Pts',(-16.7110078198973,-19.5758522575445,
-0.127175806681434));
#77856=CARTESIAN_POINT('Ctrl Pts',(-16.6890805816263,-19.5047478718232,
-0.122665413525099));
#77857=CARTESIAN_POINT('Ctrl Pts',(-16.670871275646,-19.4323727566685,-0.118155020368764));
#77858=CARTESIAN_POINT('Ctrl Pts',(-16.6565191765188,-19.3591393226743,
-0.113644627212429));
#77859=CARTESIAN_POINT('Ctrl Pts',(-16.641451763523,-19.2822559075513,-0.108909434411911));
#77860=CARTESIAN_POINT('Ctrl Pts',(-16.6306362897029,-19.2044268305763,
-0.104174241611394));
#77861=CARTESIAN_POINT('Ctrl Pts',(-16.6241750766647,-19.1261487664996,
-0.0994390488108757));
#77862=CARTESIAN_POINT('Ctrl Pts',(-16.618041066305,-19.0518347865785,-0.0949436511940506));
#77863=CARTESIAN_POINT('Ctrl Pts',(-16.6158311203138,-18.9771167035359,
-0.0904482535772255));
#77864=CARTESIAN_POINT('Ctrl Pts',(-16.6175804393308,-18.9024294117756,
-0.0859528559604003));
#77865=CARTESIAN_POINT('Ctrl Pts',(-16.6193281134804,-18.8278123477383,
-0.0814616853215709));
#77866=CARTESIAN_POINT('Ctrl Pts',(-16.6250276422425,-18.7532264655291,
-0.0769705146827415));
#77867=CARTESIAN_POINT('Ctrl Pts',(-16.6346622154624,-18.6791083247648,
-0.0724793440439121));
#77868=CARTESIAN_POINT('Ctrl Pts',(-16.6442902465126,-18.6050405124837,
-0.0679912230472238));
#77869=CARTESIAN_POINT('Ctrl Pts',(-16.6578479512151,-18.5314402553688,
-0.0635031020505355));
#77870=CARTESIAN_POINT('Ctrl Pts',(-16.6752666606882,-18.458739381659,-0.0590149810538472));
#77871=CARTESIAN_POINT('Ctrl Pts',(-16.6926780888339,-18.3860688981953,
-0.0545287361708016));
#77872=CARTESIAN_POINT('Ctrl Pts',(-16.7139472060124,-18.3142974872696,
-0.0500424912877559));
#77873=CARTESIAN_POINT('Ctrl Pts',(-16.738954437569,-18.2438459180203,-0.0455562464047103));
#77874=CARTESIAN_POINT('Ctrl Pts',(-16.7639647762088,-18.1733855953477,
-0.0410694441174684));
#77875=CARTESIAN_POINT('Ctrl Pts',(-16.7927140135935,-18.1042458686283,
-0.0365826418302264));
#77876=CARTESIAN_POINT('Ctrl Pts',(-16.8250332584604,-18.0368306278641,
-0.0320958395429845));
#77877=CARTESIAN_POINT('Ctrl Pts',(-16.8573540573157,-17.9694121456102,
-0.0276088215193051));
#77878=CARTESIAN_POINT('Ctrl Pts',(-16.893245003916,-17.9037187169574,-0.0231218034956257));
#77879=CARTESIAN_POINT('Ctrl Pts',(-16.9324905209222,-17.8401310343422,
-0.0186347854719464));
#77880=CARTESIAN_POINT('Ctrl Pts',(-16.971763121732,-17.776499469102,-0.0141446709031355));
#77881=CARTESIAN_POINT('Ctrl Pts',(-17.0143946720501,-17.7149769304511,
-0.00965455633432465));
#77882=CARTESIAN_POINT('Ctrl Pts',(-17.0601258387639,-17.65591578501,-0.00516444176551379));
#77883=CARTESIAN_POINT('Ctrl Pts',(-17.0776588692871,-17.6332721277373,
-0.00344296117700913));
#77884=CARTESIAN_POINT('Ctrl Pts',(-17.0956470822643,-17.6109899387145,
-0.00172148058850446));
#77885=CARTESIAN_POINT('Ctrl Pts',(-17.1140743056112,-17.5890877707427,
2.02192933296002E-16));
#77886=CARTESIAN_POINT('',(-20.3539400851898,-17.5891048754966,-2.19119258500671E-7));
#77887=CARTESIAN_POINT('Origin',(-18.734,-18.952,0.));
#77888=CARTESIAN_POINT('Ctrl Pts',(-20.3539400851898,-17.5891048754965,
-2.19119258500671E-7));
#77889=CARTESIAN_POINT('Ctrl Pts',(-20.3072931859159,-17.5336602703872,
-0.00438523983104841));
#77890=CARTESIAN_POINT('Ctrl Pts',(-20.2577048501402,-17.4805043431566,
-0.00877026054283832));
#77891=CARTESIAN_POINT('Ctrl Pts',(-20.2054284583706,-17.4299660674291,
-0.0131552812546282));
#77892=CARTESIAN_POINT('Ctrl Pts',(-20.1532296863998,-17.3795028307521,
-0.0175337911033991));
#77893=CARTESIAN_POINT('Ctrl Pts',(-20.0983511257708,-17.3316498632894,
-0.02191230095217));
#77894=CARTESIAN_POINT('Ctrl Pts',(-20.0410859170621,-17.2867026075148,
-0.0262908108009409));
#77895=CARTESIAN_POINT('Ctrl Pts',(-19.9838881021844,-17.2418082489151,
-0.0306641677032834));
#77896=CARTESIAN_POINT('Ctrl Pts',(-19.9243095970085,-17.1998131057542,
-0.0350375246056259));
#77897=CARTESIAN_POINT('Ctrl Pts',(-19.8626785748432,-17.1609741278558,
-0.0394108815079684));
#77898=CARTESIAN_POINT('Ctrl Pts',(-19.8010865494232,-17.1221597251417,
-0.0437814711888771));
#77899=CARTESIAN_POINT('Ctrl Pts',(-19.7374449915698,-17.0864977823033,
-0.0481520608697857));
#77900=CARTESIAN_POINT('Ctrl Pts',(-19.6721120099389,-17.054202630203,-0.0525226505506944));
#77901=CARTESIAN_POINT('Ctrl Pts',(-19.6067987309428,-17.0219172174346,
-0.0568919221816712));
#77902=CARTESIAN_POINT('Ctrl Pts',(-19.5397954737535,-16.9929967935617,
-0.061261193812648));
#77903=CARTESIAN_POINT('Ctrl Pts',(-19.471484467114,-16.9676094989228,-0.0656304654436248));
#77904=CARTESIAN_POINT('Ctrl Pts',(-19.4031714390131,-16.9422214530222,
-0.0699998663702223));
#77905=CARTESIAN_POINT('Ctrl Pts',(-19.3335510382758,-16.9203669101753,
-0.0743692672968198));
#77906=CARTESIAN_POINT('Ctrl Pts',(-19.2630233707281,-16.9021650619566,
-0.0787386682234172));
#77907=CARTESIAN_POINT('Ctrl Pts',(-19.1924239083035,-16.883944684847,-0.0831125170583778));
#77908=CARTESIAN_POINT('Ctrl Pts',(-19.1209158041551,-16.8693845460033,
-0.0874863658933384));
#77909=CARTESIAN_POINT('Ctrl Pts',(-19.0489112989914,-16.8585531117873,
-0.091860214728299));
#77910=CARTESIAN_POINT('Ctrl Pts',(-18.9768669711116,-16.8477156871527,
-0.0962364825582915));
#77911=CARTESIAN_POINT('Ctrl Pts',(-18.9043261767331,-16.8406111195394,
-0.100612750388284));
#77912=CARTESIAN_POINT('Ctrl Pts',(-18.8317055633236,-16.8372558965928,
-0.104989018218277));
#77913=CARTESIAN_POINT('Ctrl Pts',(-18.7589608117349,-16.8338949382048,
-0.109372766870793));
#77914=CARTESIAN_POINT('Ctrl Pts',(-18.6861364519369,-16.8342961174985,
-0.113756515523309));
#77915=CARTESIAN_POINT('Ctrl Pts',(-18.6136477260046,-16.8384238054558,
-0.118140264175825));
#77916=CARTESIAN_POINT('Ctrl Pts',(-18.5716413935224,-16.8408157502787,
-0.120680593048316));
#77917=CARTESIAN_POINT('Ctrl Pts',(-18.5297476644013,-16.8444581093918,
-0.123220921920807));
#77918=CARTESIAN_POINT('Ctrl Pts',(-18.4880458342194,-16.8493360828855,
-0.125761250793298));
#77919=CARTESIAN_POINT('Ctrl Pts',(-18.4158851594457,-16.8577769080795,
-0.130157025386072));
#77920=CARTESIAN_POINT('Ctrl Pts',(-18.3440241643562,-16.8699525372844,
-0.134552799978846));
#77921=CARTESIAN_POINT('Ctrl Pts',(-18.2728786958473,-16.8858305628878,
-0.138948574571619));
#77922=CARTESIAN_POINT('Ctrl Pts',(-18.2018360533927,-16.9016856400904,
-0.143337995981728));
#77923=CARTESIAN_POINT('Ctrl Pts',(-18.1315073495763,-16.9212323858817,
-0.147727417391837));
#77924=CARTESIAN_POINT('Ctrl Pts',(-18.0623020683667,-16.9443867681649,
-0.152116838801945));
#77925=CARTESIAN_POINT('Ctrl Pts',(-17.9931748039694,-16.9675150479445,
-0.156501311909554));
#77926=CARTESIAN_POINT('Ctrl Pts',(-17.9251688996743,-16.9942427328983,
-0.160885785017163));
#77927=CARTESIAN_POINT('Ctrl Pts',(-17.8586807914584,-17.0244354010415,
-0.165270258124772));
#77928=CARTESIAN_POINT('Ctrl Pts',(-17.7922329666599,-17.0546097762315,
-0.169652074794037));
#77929=CARTESIAN_POINT('Ctrl Pts',(-17.7273015495518,-17.088244770482,-0.174033891463303));
#77930=CARTESIAN_POINT('Ctrl Pts',(-17.664263699225,-17.1251575747197,-0.178415708132568));
#77931=CARTESIAN_POINT('Ctrl Pts',(-17.601243455081,-17.1620600693801,-0.182796300980502));
#77932=CARTESIAN_POINT('Ctrl Pts',(-17.5401161419552,-17.2022383136031,
-0.187176893828435));
#77933=CARTESIAN_POINT('Ctrl Pts',(-17.481233502117,-17.2454640051315,-0.191557486676369));
#77934=CARTESIAN_POINT('Ctrl Pts',(-17.4223480788122,-17.2886917400001,
-0.195938286601192));
#77935=CARTESIAN_POINT('Ctrl Pts',(-17.3657079255823,-17.3349669223205,
-0.200319086526015));
#77936=CARTESIAN_POINT('Ctrl Pts',(-17.3116336689764,-17.3840194451555,
-0.204699886450839));
#77937=CARTESIAN_POINT('Ctrl Pts',(-17.2575022929462,-17.4331237828844,
-0.20908531387839));
#77938=CARTESIAN_POINT('Ctrl Pts',(-17.2059425814251,-17.4850109948883,
-0.213470741305941));
#77939=CARTESIAN_POINT('Ctrl Pts',(-17.1572394598231,-17.5393729441424,
-0.217856168733492));
#77940=CARTESIAN_POINT('Ctrl Pts',(-17.1085090930288,-17.5937653042143,
-0.222244049429123));
#77941=CARTESIAN_POINT('Ctrl Pts',(-17.0626387997765,-17.6506347838423,
-0.226631930124753));
#77942=CARTESIAN_POINT('Ctrl Pts',(-17.019872504564,-17.7096409820867,-0.231019810820383));
#77943=CARTESIAN_POINT('Ctrl Pts',(-16.9770304728485,-17.7687516767129,
-0.235415462185369));
#77944=CARTESIAN_POINT('Ctrl Pts',(-16.9373036781403,-17.8300062430901,
-0.239811113550354));
#77945=CARTESIAN_POINT('Ctrl Pts',(-16.9008917879239,-17.8930366942999,
-0.24420676491534));
#77946=CARTESIAN_POINT('Ctrl Pts',(-16.8767856560651,-17.9347653812468,
-0.247116862435137));
#77947=CARTESIAN_POINT('Ctrl Pts',(-16.8541314891368,-17.9772719122011,
-0.250026959954935));
#77948=CARTESIAN_POINT('Ctrl Pts',(-16.8329756005513,-18.0204447237546,
-0.252937057474732));
#77949=CARTESIAN_POINT('Ctrl Pts',(-16.8011149915786,-18.0854626529992,
-0.257319642435692));
#77950=CARTESIAN_POINT('Ctrl Pts',(-16.7725300877984,-18.1522470560443,
-0.261702227396653));
#77951=CARTESIAN_POINT('Ctrl Pts',(-16.7474199512368,-18.2204340700553,
-0.266084812357613));
#77952=CARTESIAN_POINT('Ctrl Pts',(-16.7223475943392,-18.2885184927293,
-0.27046080346405));
#77953=CARTESIAN_POINT('Ctrl Pts',(-16.7007397931117,-18.3580008874103,
-0.274836794570486));
#77954=CARTESIAN_POINT('Ctrl Pts',(-16.6827489310325,-18.4284944584252,
-0.279212785676922));
#77955=CARTESIAN_POINT('Ctrl Pts',(-16.6647796228869,-18.4989035746903,
-0.283583534131739));
#77956=CARTESIAN_POINT('Ctrl Pts',(-16.6504187653927,-18.5703209945558,
-0.287954282586557));
#77957=CARTESIAN_POINT('Ctrl Pts',(-16.6397694152316,-18.6423433226609,
-0.292325031041374));
#77958=CARTESIAN_POINT('Ctrl Pts',(-16.6291269614596,-18.714319009986,-0.296692949052881));
#77959=CARTESIAN_POINT('Ctrl Pts',(-16.6221913171743,-18.7868983510167,
-0.301060867064388));
#77960=CARTESIAN_POINT('Ctrl Pts',(-16.6190144817355,-18.8596676788374,
-0.305428785075896));
#77961=CARTESIAN_POINT('Ctrl Pts',(-16.6158386481743,-18.9324140574164,
-0.309795325578372));
#77962=CARTESIAN_POINT('Ctrl Pts',(-16.616419291388,-19.0053498208129,-0.314161866080849));
#77963=CARTESIAN_POINT('Ctrl Pts',(-16.6207564193529,-19.0780577996553,
-0.318528406583326));
#77964=CARTESIAN_POINT('Ctrl Pts',(-16.6250936203624,-19.1507670030232,
-0.322895020625736));
#77965=CARTESIAN_POINT('Ctrl Pts',(-16.6331874009118,-19.2232479313927,
-0.327261634668147));
#77966=CARTESIAN_POINT('Ctrl Pts',(-16.6449857626134,-19.2950867470421,
-0.331628248710558));
#77967=CARTESIAN_POINT('Ctrl Pts',(-16.6567963363639,-19.3669999203992,
-0.335999382474065));
#77968=CARTESIAN_POINT('Ctrl Pts',(-16.6723190685484,-19.4382691756095,
-0.340370516237573));
#77969=CARTESIAN_POINT('Ctrl Pts',(-16.6914506293117,-19.5084899534591,
-0.34474165000108));
#77970=CARTESIAN_POINT('Ctrl Pts',(-16.7105925668403,-19.578748818349,-0.349115154623359));
#77971=CARTESIAN_POINT('Ctrl Pts',(-16.7333470785607,-19.6479576138077,
-0.353488659245638));
#77972=CARTESIAN_POINT('Ctrl Pts',(-16.7595614725531,-19.715728683063,-0.357862163867917));
#77973=CARTESIAN_POINT('Ctrl Pts',(-16.7858226024992,-19.7836205769906,
-0.362243465729766));
#77974=CARTESIAN_POINT('Ctrl Pts',(-16.815555734801,-19.8500691841256,-0.366624767591615));
#77975=CARTESIAN_POINT('Ctrl Pts',(-16.8485609817508,-19.9147090466302,
-0.371006069453464));
#77976=CARTESIAN_POINT('Ctrl Pts',(-16.871428766834,-19.9594949706928,-0.374041667687698));
#77977=CARTESIAN_POINT('Ctrl Pts',(-16.8958663395961,-20.0034131234881,
-0.377077265921932));
#77978=CARTESIAN_POINT('Ctrl Pts',(-16.9217951774031,-20.0463503465328,
-0.380112864156166));
#77979=CARTESIAN_POINT('Ctrl Pts',(-16.9592871194148,-20.108435654348,-0.384502203694482));
#77980=CARTESIAN_POINT('Ctrl Pts',(-17.0000462087351,-20.1687128298791,
-0.388891543232798));
#77981=CARTESIAN_POINT('Ctrl Pts',(-17.0438726579669,-20.2268170722547,
-0.393280882771115));
#77982=CARTESIAN_POINT('Ctrl Pts',(-17.0876341208282,-20.2848351569816,
-0.39766371374554));
#77983=CARTESIAN_POINT('Ctrl Pts',(-17.1344536264988,-20.3406863231545,
-0.402046544719966));
#77984=CARTESIAN_POINT('Ctrl Pts',(-17.1840869213949,-20.3940327488545,
-0.406429375694392));
#77985=CARTESIAN_POINT('Ctrl Pts',(-17.233661916773,-20.4473165135744,-0.410807058573503));
#77986=CARTESIAN_POINT('Ctrl Pts',(-17.286043808912,-20.4981010311795,-0.415184741452614));
#77987=CARTESIAN_POINT('Ctrl Pts',(-17.3409477702608,-20.5460810786214,
-0.419562424331725));
#77988=CARTESIAN_POINT('Ctrl Pts',(-17.3958169194767,-20.5940307040728,
-0.423937331518979));
#77989=CARTESIAN_POINT('Ctrl Pts',(-17.4532046028362,-20.6391790711338,
-0.428312238706232));
#77990=CARTESIAN_POINT('Ctrl Pts',(-17.512789805683,-20.6812584136838,-0.432687145893485));
#77991=CARTESIAN_POINT('Ctrl Pts',(-17.5723568562233,-20.7233249369921,
-0.437060720289174));
#77992=CARTESIAN_POINT('Ctrl Pts',(-17.6341197035788,-20.7623240140803,
-0.441434294684862));
#77993=CARTESIAN_POINT('Ctrl Pts',(-17.6977263244878,-20.7980297585468,
-0.44580786908055));
#77994=CARTESIAN_POINT('Ctrl Pts',(-17.7613345200932,-20.8337363869733,
-0.450181551751953));
#77995=CARTESIAN_POINT('Ctrl Pts',(-17.8267861585153,-20.8661492866598,
-0.454555234423356));
#77996=CARTESIAN_POINT('Ctrl Pts',(-17.893703933171,-20.8950881400677,-0.458928917094759));
#77997=CARTESIAN_POINT('Ctrl Pts',(-17.9606909349874,-20.9240569310321,
-0.463307124388127));
#77998=CARTESIAN_POINT('Ctrl Pts',(-18.0291466578796,-20.9495443083808,
-0.467685331681495));
#77999=CARTESIAN_POINT('Ctrl Pts',(-18.0986738647243,-20.9714181592319,
-0.472063538974863));
#78000=CARTESIAN_POINT('Ctrl Pts',(-18.168238941735,-20.9933039243595,-0.476444130995652));
#78001=CARTESIAN_POINT('Ctrl Pts',(-18.2388761976448,-21.0115721233672,
-0.480824723016442));
#78002=CARTESIAN_POINT('Ctrl Pts',(-18.3101759171464,-21.026141303478,-0.485205315037232));
#78003=CARTESIAN_POINT('Ctrl Pts',(-18.381601628856,-21.040736228475,-0.4895936479084));
#78004=CARTESIAN_POINT('Ctrl Pts',(-18.4536916647472,-21.0516190094181,
-0.493981980779569));
#78005=CARTESIAN_POINT('Ctrl Pts',(-18.5260294507968,-21.0587598939281,
-0.498370313650738));
#78006=CARTESIAN_POINT('Ctrl Pts',(-18.5750331942105,-21.063597339078,-0.501343099379692));
#78007=CARTESIAN_POINT('Ctrl Pts',(-18.6241505410346,-21.0667186770647,
-0.504315885108646));
#78008=CARTESIAN_POINT('Ctrl Pts',(-18.6732524746729,-21.0681282423725,
-0.5072886708376));
#78009=CARTESIAN_POINT('Ctrl Pts',(-18.7457477477536,-21.0702093584171,
-0.511677763023227));
#78010=CARTESIAN_POINT('Ctrl Pts',(-18.8184909227825,-21.068564845846,-0.516066855208853));
#78011=CARTESIAN_POINT('Ctrl Pts',(-18.8910671418926,-21.063165297398,-0.520455947394479));
#78012=CARTESIAN_POINT('Ctrl Pts',(-18.9635359951035,-21.0577737367921,
-0.524838546560291));
#78013=CARTESIAN_POINT('Ctrl Pts',(-19.035837905828,-21.0486382034475,-0.529221145726102));
#78014=CARTESIAN_POINT('Ctrl Pts',(-19.1075566421874,-21.0357812829272,
-0.533603744891914));
#78015=CARTESIAN_POINT('Ctrl Pts',(-19.1791915341236,-21.0229393930828,
-0.537981220480295));
#78016=CARTESIAN_POINT('Ctrl Pts',(-19.2502441338016,-21.0063848432238,
-0.542358696068677));
#78017=CARTESIAN_POINT('Ctrl Pts',(-19.32030366582,-20.9861919799876,-0.546736171657058));
#78018=CARTESIAN_POINT('Ctrl Pts',(-19.3903190177729,-20.9660118505222,
-0.551110886776556));
#78019=CARTESIAN_POINT('Ctrl Pts',(-19.4593420824551,-20.9421980932421,
-0.555485601896053));
#78020=CARTESIAN_POINT('Ctrl Pts',(-19.5269740036053,-20.91487575501,-0.559860317015551));
#78021=CARTESIAN_POINT('Ctrl Pts',(-19.5945855605349,-20.8875616436346,
-0.564233714892222));
#78022=CARTESIAN_POINT('Ctrl Pts',(-19.6608063587657,-20.8567412292127,
-0.568607112768892));
#78023=CARTESIAN_POINT('Ctrl Pts',(-19.7252559833366,-20.8225882966328,
-0.572980510645563));
#78024=CARTESIAN_POINT('Ctrl Pts',(-19.7897074377076,-20.7884343944112,
-0.577354032688112));
#78025=CARTESIAN_POINT('Ctrl Pts',(-19.8523871934859,-20.750948013708,-0.581727554730662));
#78026=CARTESIAN_POINT('Ctrl Pts',(-19.91293947795,-20.7103488582563,-0.586101076773212));
#78027=CARTESIAN_POINT('Ctrl Pts',(-19.973554763754,-20.6697074616039,-0.590479149226235));
#78028=CARTESIAN_POINT('Ctrl Pts',(-20.0320377575058,-20.6259470930868,
-0.594857221679259));
#78029=CARTESIAN_POINT('Ctrl Pts',(-20.0880624400642,-20.5793303009554,
-0.599235294132282));
#78030=CARTESIAN_POINT('Ctrl Pts',(-20.144117821258,-20.532687965227,-0.603615765543122));
#78031=CARTESIAN_POINT('Ctrl Pts',(-20.1977118548976,-20.4831864169908,
-0.607996236953962));
#78032=CARTESIAN_POINT('Ctrl Pts',(-20.2485543758913,-20.4311261076962,
-0.612376708364801));
#78033=CARTESIAN_POINT('Ctrl Pts',(-20.2994870261127,-20.3789735103841,
-0.616764945096826));
#78034=CARTESIAN_POINT('Ctrl Pts',(-20.3476581043646,-20.3242534561184,
-0.62115318182885));
#78035=CARTESIAN_POINT('Ctrl Pts',(-20.3928172134661,-20.2673001377285,
-0.625541418560875));
#78036=CARTESIAN_POINT('Ctrl Pts',(-20.4234261206891,-20.2286970989767,
-0.628515771546929));
#78037=CARTESIAN_POINT('Ctrl Pts',(-20.4526521510532,-20.1890687322311,
-0.631490124532982));
#78038=CARTESIAN_POINT('Ctrl Pts',(-20.4804290435443,-20.1485260531492,
-0.634464477519035));
#78039=CARTESIAN_POINT('Ctrl Pts',(-20.5219934354816,-20.0878593747552,
-0.6389151976027));
#78040=CARTESIAN_POINT('Ctrl Pts',(-20.5604705838686,-20.0249114796293,
-0.643365917686366));
#78041=CARTESIAN_POINT('Ctrl Pts',(-20.5956057938581,-19.9600242399239,
-0.647816637770031));
#78042=CARTESIAN_POINT('Ctrl Pts',(-20.6306759070159,-19.8952572201836,
-0.652259111773021));
#78043=CARTESIAN_POINT('Ctrl Pts',(-20.6624161699,-19.8285584030127,-0.656701585776012));
#78044=CARTESIAN_POINT('Ctrl Pts',(-20.6906149824499,-19.760298713628,-0.661144059779002));
#78045=CARTESIAN_POINT('Ctrl Pts',(-20.7018340510959,-19.7331411820968,
-0.662911525012145));
#78046=CARTESIAN_POINT('Ctrl Pts',(-20.7124930319529,-19.7057368944626,
-0.664678990245288));
#78047=CARTESIAN_POINT('Ctrl Pts',(-20.7225805821191,-19.6781103693095,
-0.666446455478431));
#78048=CARTESIAN_POINT('Origin',(18.734,-18.952,0.));
#78049=CARTESIAN_POINT('',(16.745419449923,-19.6781104570625,-21.2464098137458));
#78050=CARTESIAN_POINT('',(16.7454194499919,-19.678110457251,-21.4658225324418));
#78051=CARTESIAN_POINT('',(16.7454194499637,-19.6781104571739,0.));
#78052=CARTESIAN_POINT('',(16.6170006158577,-18.953614788214,-21.5109437210328));
#78053=CARTESIAN_POINT('Ctrl Pts',(16.7454194499919,-19.678110457251,-21.4658225324418));
#78054=CARTESIAN_POINT('Ctrl Pts',(16.7444838645978,-19.6755481929303,-21.4659708416694));
#78055=CARTESIAN_POINT('Ctrl Pts',(16.7435532220733,-19.672984094887,-21.466119187511));
#78056=CARTESIAN_POINT('Ctrl Pts',(16.7287348633895,-19.6319093107387,-21.4684945478173));
#78057=CARTESIAN_POINT('Ctrl Pts',(16.7159624561017,-19.5930064377761,-21.4707298068511));
#78058=CARTESIAN_POINT('Ctrl Pts',(16.6989527891759,-19.5356344857477,-21.4740350315673));
#78059=CARTESIAN_POINT('Ctrl Pts',(16.6938224023506,-19.5174393926652,-21.4750845544372));
#78060=CARTESIAN_POINT('Ctrl Pts',(16.67330414272,-19.4407529854473,-21.479522275393));
#78061=CARTESIAN_POINT('Ctrl Pts',(16.6601842244916,-19.3816901056815,-21.4829746671899));
#78062=CARTESIAN_POINT('Ctrl Pts',(16.6480276539524,-19.3132345736383,-21.4870987991129));
#78063=CARTESIAN_POINT('Ctrl Pts',(16.6465011846899,-19.3043063086001,-21.4876390674732));
#78064=CARTESIAN_POINT('Ctrl Pts',(16.644305726321,-19.2909496980064,-21.4884512303201));
#78065=CARTESIAN_POINT('Ctrl Pts',(16.6435933949815,-19.286528444333,-21.4887207108556));
#78066=CARTESIAN_POINT('Ctrl Pts',(16.6423404404213,-19.2785913960363,-21.4892056875075));
#78067=CARTESIAN_POINT('Ctrl Pts',(16.6417946456356,-19.2750764736216,-21.4894208862796));
#78068=CARTESIAN_POINT('Ctrl Pts',(16.6407480030303,-19.2682221989107,-21.4898413667536));
#78069=CARTESIAN_POINT('Ctrl Pts',(16.640246287296,-19.2648830325719,-21.4900465921491));
#78070=CARTESIAN_POINT('Ctrl Pts',(16.6391505446239,-19.2574696572128,-21.4905030441399));
#78071=CARTESIAN_POINT('Ctrl Pts',(16.6385604120744,-19.2533948985467,-21.4907544855749));
#78072=CARTESIAN_POINT('Ctrl Pts',(16.637120554269,-19.2432442762658,-21.4913821828982));
#78073=CARTESIAN_POINT('Ctrl Pts',(16.6362853529834,-19.2371664356149,-21.4917592136064));
#78074=CARTESIAN_POINT('Ctrl Pts',(16.6323978968592,-19.2079355069642,-21.4935779411442));
#78075=CARTESIAN_POINT('Ctrl Pts',(16.6297026110604,-19.1847375792239,-21.4950376377215));
#78076=CARTESIAN_POINT('Ctrl Pts',(16.6205187442238,-19.0923904497098,-21.5009009048513));
#78077=CARTESIAN_POINT('Ctrl Pts',(16.6170514757345,-19.0229900275189,-21.5054225881123));
#78078=CARTESIAN_POINT('Ctrl Pts',(16.6170005689161,-18.9535520277953,-21.5099894676286));
#78079=CARTESIAN_POINT('',(20.3539256943886,-20.3149122292574,-22.));
#78080=CARTESIAN_POINT('Ctrl Pts',(16.6170006158577,-18.953614788214,-21.5109437210328));
#78081=CARTESIAN_POINT('Ctrl Pts',(16.6169439842755,-18.879370361958,-21.5154240901546));
#78082=CARTESIAN_POINT('Ctrl Pts',(16.620797918379,-18.8049814529217,-21.5199044592764));
#78083=CARTESIAN_POINT('Ctrl Pts',(16.6285774617411,-18.730900621006,-21.5243848283982));
#78084=CARTESIAN_POINT('Ctrl Pts',(16.6360763262784,-18.6594925578986,-21.5287035498909));
#78085=CARTESIAN_POINT('Ctrl Pts',(16.6472223388839,-18.5883712693749,-21.5330222713836));
#78086=CARTESIAN_POINT('Ctrl Pts',(16.6619760550115,-18.5179426634713,-21.5373409928764));
#78087=CARTESIAN_POINT('Ctrl Pts',(16.6767199425897,-18.4475609753088,-21.541656837347));
#78088=CARTESIAN_POINT('Ctrl Pts',(16.6950666675508,-18.3778715396864,-21.5459726818176));
#78089=CARTESIAN_POINT('Ctrl Pts',(16.7169252861184,-18.3092725316128,-21.5502885262882));
#78090=CARTESIAN_POINT('Ctrl Pts',(16.738777013927,-18.2406951488414,-21.5546030102225));
#78091=CARTESIAN_POINT('Ctrl Pts',(16.7641382879759,-18.1732079844748,-21.5589174941569));
#78092=CARTESIAN_POINT('Ctrl Pts',(16.792868144003,-18.1071946273647,-21.5632319780912));
#78093=CARTESIAN_POINT('Ctrl Pts',(16.8215990247681,-18.0411789156865,-21.5675466159148));
#78094=CARTESIAN_POINT('Ctrl Pts',(16.8536985247398,-17.9766375696395,-21.5718612537383));
#78095=CARTESIAN_POINT('Ctrl Pts',(16.8889780706294,-17.9139330078739,-21.5761758915619));
#78096=CARTESIAN_POINT('Ctrl Pts',(16.9242925056221,-17.8511664355052,-21.5804947962727));
#78097=CARTESIAN_POINT('Ctrl Pts',(16.9627930151098,-17.7902407038457,-21.5848137009835));
#78098=CARTESIAN_POINT('Ctrl Pts',(17.0042462802129,-17.7314914711963,-21.5891326056943));
#78099=CARTESIAN_POINT('Ctrl Pts',(17.0457242009246,-17.6727072956277,-21.593454079207));
#78100=CARTESIAN_POINT('Ctrl Pts',(17.0901580619222,-17.6161025825292,-21.5977755527196));
#78101=CARTESIAN_POINT('Ctrl Pts',(17.1372743754074,-17.5619797556261,-21.6020970262323));
#78102=CARTESIAN_POINT('Ctrl Pts',(17.1844652778813,-17.5077712478488,-21.606425340992));
#78103=CARTESIAN_POINT('Ctrl Pts',(17.2343467552723,-17.4560528156038,-21.6107536557517));
#78104=CARTESIAN_POINT('Ctrl Pts',(17.2866094559726,-17.4070891245576,-21.6150819705114));
#78105=CARTESIAN_POINT('Ctrl Pts',(17.3002562150789,-17.3943037979728,-21.6162121736595));
#78106=CARTESIAN_POINT('Ctrl Pts',(17.3140651673995,-17.3817060763086,-21.6173423768076));
#78107=CARTESIAN_POINT('Ctrl Pts',(17.3280304696825,-17.3693001927659,-21.6184725799558));
#78108=CARTESIAN_POINT('Ctrl Pts',(17.3823193529476,-17.3210734125788,-21.6228661452028));
#78109=CARTESIAN_POINT('Ctrl Pts',(17.4391955190593,-17.2755515953447,-21.6272597104498));
#78110=CARTESIAN_POINT('Ctrl Pts',(17.4983586556721,-17.2330237150596,-21.6316532756968));
#78111=CARTESIAN_POINT('Ctrl Pts',(17.5574354931409,-17.1905578686671,-21.6360404322079));
#78112=CARTESIAN_POINT('Ctrl Pts',(17.6187922908035,-17.1510775674503,-21.640427588719));
#78113=CARTESIAN_POINT('Ctrl Pts',(17.6820943811751,-17.1148327324153,-21.64481474523));
#78114=CARTESIAN_POINT('Ctrl Pts',(17.7453240043386,-17.0786293898806,-21.6491968793954));
#78115=CARTESIAN_POINT('Ctrl Pts',(17.810494080778,-17.0456543930935,-21.6535790135607));
#78116=CARTESIAN_POINT('Ctrl Pts',(17.8772409624661,-17.0161144270376,-21.6579611477261));
#78117=CARTESIAN_POINT('Ctrl Pts',(17.9439467029022,-16.9865926687415,-21.6623405808441));
#78118=CARTESIAN_POINT('Ctrl Pts',(18.0122268812651,-16.9605019339683,-21.6667200139621));
#78119=CARTESIAN_POINT('Ctrl Pts',(18.0816945039053,-16.9380023486199,-21.6710994470801));
#78120=CARTESIAN_POINT('Ctrl Pts',(18.1511420514884,-16.9155092652999,-21.6754776146104));
#78121=CARTESIAN_POINT('Ctrl Pts',(18.2217759047592,-16.8966054189395,-21.6798557821407));
#78122=CARTESIAN_POINT('Ctrl Pts',(18.2931919729642,-16.881401708853,-21.684233949671));
#78123=CARTESIAN_POINT('Ctrl Pts',(18.364610783359,-16.866197414984,-21.6886122853114));
#78124=CARTESIAN_POINT('Ctrl Pts',(18.4368113975566,-16.8546936376761,-21.6929906209519));
#78125=CARTESIAN_POINT('Ctrl Pts',(18.5093791774671,-16.8469502414231,-21.6973689565923));
#78126=CARTESIAN_POINT('Ctrl Pts',(18.5820229096485,-16.8391987406294,-21.7017518747697));
#78127=CARTESIAN_POINT('Ctrl Pts',(18.6550340955975,-16.8352155299105,-21.7061347929472));
#78128=CARTESIAN_POINT('Ctrl Pts',(18.7279934268567,-16.835008521255,-21.7105177111246));
#78129=CARTESIAN_POINT('Ctrl Pts',(18.8009931127498,-16.8348013981006,-21.7149030535438));
#78130=CARTESIAN_POINT('Ctrl Pts',(18.8739404062014,-16.8383746122317,-21.719288395963));
#78131=CARTESIAN_POINT('Ctrl Pts',(18.9464191616025,-16.845683998118,-21.7236737383821));
#78132=CARTESIAN_POINT('Ctrl Pts',(19.019026007826,-16.8530063017931,-21.7280668309636));
#78133=CARTESIAN_POINT('Ctrl Pts',(19.0911621866738,-16.8640778900689,-21.7324599235451));
#78134=CARTESIAN_POINT('Ctrl Pts',(19.1624203793687,-16.8788031983091,-21.7368530161266));
#78135=CARTESIAN_POINT('Ctrl Pts',(19.2099755048328,-16.8886303333286,-21.7397848062968));
#78136=CARTESIAN_POINT('Ctrl Pts',(19.2571398375277,-16.9000836817304,-21.742716596467));
#78137=CARTESIAN_POINT('Ctrl Pts',(19.3037965853284,-16.9131226492631,-21.7456483866372));
#78138=CARTESIAN_POINT('Ctrl Pts',(19.3728941566259,-16.932433060537,-21.7499903005052));
#78139=CARTESIAN_POINT('Ctrl Pts',(19.4411600971652,-16.9553024383045,-21.7543322143732));
#78140=CARTESIAN_POINT('Ctrl Pts',(19.5081957188875,-16.9816421673066,-21.7586741282413));
#78141=CARTESIAN_POINT('Ctrl Pts',(19.5751303969638,-17.007942233392,-21.7630095039643));
#78142=CARTESIAN_POINT('Ctrl Pts',(19.6408379766924,-17.0377021052713,-21.7673448796873));
#78143=CARTESIAN_POINT('Ctrl Pts',(19.7049332499917,-17.0707829407374,-21.7716802554104));
#78144=CARTESIAN_POINT('Ctrl Pts',(19.7689548569736,-17.1038257555634,-21.7760106483765));
#78145=CARTESIAN_POINT('Ctrl Pts',(19.8313673996942,-17.1401817328403,-21.7803410413427));
#78146=CARTESIAN_POINT('Ctrl Pts',(19.8918057405323,-17.1796640083804,-21.7846714343088));
#78147=CARTESIAN_POINT('Ctrl Pts',(19.9522069377095,-17.2191220192527,-21.7889991659403));
#78148=CARTESIAN_POINT('Ctrl Pts',(20.0106359263449,-17.2617022501812,-21.7933268975719));
#78149=CARTESIAN_POINT('Ctrl Pts',(20.0667536873044,-17.307172772302,-21.7976546292034));
#78150=CARTESIAN_POINT('Ctrl Pts',(20.1228564014125,-17.3526311024149,-21.8019812004406));
#78151=CARTESIAN_POINT('Ctrl Pts',(20.1766487340221,-17.4009778759096,-21.8063077716777));
#78152=CARTESIAN_POINT('Ctrl Pts',(20.2278235795987,-17.4519399635232,-21.8106343429149));
#78153=CARTESIAN_POINT('Ctrl Pts',(20.2790024328481,-17.5029060421478,-21.8149612529802));
#78154=CARTESIAN_POINT('Ctrl Pts',(20.3275630441483,-17.5564874916594,-21.8192881630456));
#78155=CARTESIAN_POINT('Ctrl Pts',(20.3732354326212,-17.6123746059293,-21.823615073111));
#78156=CARTESIAN_POINT('Ctrl Pts',(20.4189626303271,-17.6683287876325,-21.8279471756927));
#78157=CARTESIAN_POINT('Ctrl Pts',(20.4617943736678,-17.7265937742531,-21.8322792782743));
#78158=CARTESIAN_POINT('Ctrl Pts',(20.5015018190868,-17.7868277725912,-21.836611380856));
#78159=CARTESIAN_POINT('Ctrl Pts',(20.5412337707152,-17.8470989454934,-21.8409461570777));
#78160=CARTESIAN_POINT('Ctrl Pts',(20.5778373403004,-17.9093411211074,-21.8452809332993));
#78161=CARTESIAN_POINT('Ctrl Pts',(20.6111293159145,-17.973187182688,-21.8496157095209));
#78162=CARTESIAN_POINT('Ctrl Pts',(20.6444883378172,-18.0371618230444,-21.8539592154936));
#78163=CARTESIAN_POINT('Ctrl Pts',(20.674522245953,-18.1027463491743,-21.8583027214662));
#78164=CARTESIAN_POINT('Ctrl Pts',(20.7010959324481,-18.1695534570681,-21.8626462274389));
#78165=CARTESIAN_POINT('Ctrl Pts',(20.7218522888838,-18.2217356089171,-21.8660388827321));
#78166=CARTESIAN_POINT('Ctrl Pts',(20.7404985496073,-18.2746632207694,-21.8694315380253));
#78167=CARTESIAN_POINT('Ctrl Pts',(20.7569919383483,-18.3281469585088,-21.8728241933186));
#78168=CARTESIAN_POINT('Ctrl Pts',(20.7789191314163,-18.3992510998001,-21.8773345707065));
#78169=CARTESIAN_POINT('Ctrl Pts',(20.7971284192367,-18.4716259697097,-21.8818449480945));
#78170=CARTESIAN_POINT('Ctrl Pts',(20.8114805262578,-18.5448591607076,-21.8863553254824));
#78171=CARTESIAN_POINT('Ctrl Pts',(20.8265480064888,-18.621742621512,-21.891090520254));
#78172=CARTESIAN_POINT('Ctrl Pts',(20.8373635429458,-18.6995717540552,-21.8958257150255));
#78173=CARTESIAN_POINT('Ctrl Pts',(20.843824811693,-18.7778498809511,-21.9005609097971));
#78174=CARTESIAN_POINT('Ctrl Pts',(20.8499588507186,-18.8521636270621,-21.9050562915339));
#78175=CARTESIAN_POINT('Ctrl Pts',(20.8521688501583,-18.9268814796183,-21.9095516732707));
#78176=CARTESIAN_POINT('Ctrl Pts',(20.8504196084828,-19.0015685467751,-21.9140470550075));
#78177=CARTESIAN_POINT('Ctrl Pts',(20.8486720115918,-19.0761853868609,-21.9185382098078));
#78178=CARTESIAN_POINT('Ctrl Pts',(20.8429725838885,-19.1507710509859,-21.9230293646081));
#78179=CARTESIAN_POINT('Ctrl Pts',(20.8333381346341,-19.2248889819521,-21.9275205194084));
#78180=CARTESIAN_POINT('Ctrl Pts',(20.8237102273003,-19.2989565858473,-21.9320086246542));
#78181=CARTESIAN_POINT('Ctrl Pts',(20.8101526690551,-19.3725566428308,-21.9364967299001));
#78182=CARTESIAN_POINT('Ctrl Pts',(20.7927341278966,-19.4452573269945,-21.9409848351459));
#78183=CARTESIAN_POINT('Ctrl Pts',(20.7753228675005,-19.5179276230559,-21.9454710644121));
#78184=CARTESIAN_POINT('Ctrl Pts',(20.7540539396924,-19.5896988571003,-21.9499572936783));
#78185=CARTESIAN_POINT('Ctrl Pts',(20.7290469182522,-19.6601502622835,-21.9544435229445));
#78186=CARTESIAN_POINT('Ctrl Pts',(20.7040367879202,-19.7306104260392,-21.9589303099422));
#78187=CARTESIAN_POINT('Ctrl Pts',(20.6752877790479,-19.7997500064623,-21.9634170969398));
#78188=CARTESIAN_POINT('Ctrl Pts',(20.6429687820359,-19.8671651158193,-21.9679038839375));
#78189=CARTESIAN_POINT('Ctrl Pts',(20.6106482296079,-19.9345834696624,-21.9723908868707));
#78190=CARTESIAN_POINT('Ctrl Pts',(20.5747575484645,-20.0002767846379,-21.9768778898039));
#78191=CARTESIAN_POINT('Ctrl Pts',(20.5355123150534,-20.0638643706455,-21.9813648927371));
#78192=CARTESIAN_POINT('Ctrl Pts',(20.4962399941625,-20.1274958454851,-21.9858549926477));
#78193=CARTESIAN_POINT('Ctrl Pts',(20.4536087412679,-20.1890183104101,-21.9903450925584));
#78194=CARTESIAN_POINT('Ctrl Pts',(20.407877888554,-20.2480794011981,-21.994835192469));
#78195=CARTESIAN_POINT('Ctrl Pts',(20.3903436794274,-20.2707247151527,-21.9965567949793));
#78196=CARTESIAN_POINT('Ctrl Pts',(20.372354222822,-20.2930085100904,-21.9982783974897));
#78197=CARTESIAN_POINT('Ctrl Pts',(20.3539256943887,-20.3149122292573,-22.));
#78198=CARTESIAN_POINT('',(17.1140599642913,-20.3148951833168,-21.9999997809128));
#78199=CARTESIAN_POINT('Origin',(18.734,-18.952,-22.));
#78200=CARTESIAN_POINT('',(16.6170002905213,-18.9531090839331,-21.2890562790225));
#78201=CARTESIAN_POINT('Ctrl Pts',(17.1140599642913,-20.3148951833168,-21.9999997809128));
#78202=CARTESIAN_POINT('Ctrl Pts',(17.1607068994597,-20.3703398270043,-21.9956147572469));
#78203=CARTESIAN_POINT('Ctrl Pts',(17.210295274204,-20.4234957880638,-21.9912297335811));
#78204=CARTESIAN_POINT('Ctrl Pts',(17.2625717073312,-20.4740340927633,-21.9868447099152));
#78205=CARTESIAN_POINT('Ctrl Pts',(17.3147705210273,-20.5244973587843,-21.9824661970807));
#78206=CARTESIAN_POINT('Ctrl Pts',(17.3696491258074,-20.5723503507068,-21.9780876842462));
#78207=CARTESIAN_POINT('Ctrl Pts',(17.4269143804502,-20.6172976260014,-21.9737091714118));
#78208=CARTESIAN_POINT('Ctrl Pts',(17.4841122416856,-20.6621920044732,-21.9693358114907));
#78209=CARTESIAN_POINT('Ctrl Pts',(17.5436907950378,-20.7041871625307,-21.9649624515697));
#78210=CARTESIAN_POINT('Ctrl Pts',(17.605321866596,-20.7430261503327,-21.9605890916486));
#78211=CARTESIAN_POINT('Ctrl Pts',(17.6669139416705,-20.7818405631288,-21.9562184989301));
#78212=CARTESIAN_POINT('Ctrl Pts',(17.7305555504131,-20.8175025110335,-21.9518479062116));
#78213=CARTESIAN_POINT('Ctrl Pts',(17.7958885836047,-20.8497976631951,-21.9474773134931));
#78214=CARTESIAN_POINT('Ctrl Pts',(17.8612019143776,-20.8820830761394,-21.94310803881));
#78215=CARTESIAN_POINT('Ctrl Pts',(17.9282052240273,-20.9110034951629,-21.9387387641268));
#78216=CARTESIAN_POINT('Ctrl Pts',(17.9965162832812,-20.9363907799561,-21.9343694894437));
#78217=CARTESIAN_POINT('Ctrl Pts',(18.0648293641575,-20.9617788160697,-21.9300000854546));
#78218=CARTESIAN_POINT('Ctrl Pts',(18.1344498178311,-20.9836333441171,-21.9256306814655));
#78219=CARTESIAN_POINT('Ctrl Pts',(18.2049775379727,-21.0018351725616,-21.9212612774765));
#78220=CARTESIAN_POINT('Ctrl Pts',(18.2755770529193,-21.0200555298444,-21.9168874255837));
#78221=CARTESIAN_POINT('Ctrl Pts',(18.347085209244,-21.0346156438901,-21.912513573691));
#78222=CARTESIAN_POINT('Ctrl Pts',(18.4190897657556,-21.0454470483793,-21.9081397217982));
#78223=CARTESIAN_POINT('Ctrl Pts',(18.4911341450163,-21.0562844432714,-21.9037634509084));
#78224=CARTESIAN_POINT('Ctrl Pts',(18.5636749899472,-21.0633889762076,-21.8993871800187));
#78225=CARTESIAN_POINT('Ctrl Pts',(18.6362956526055,-21.0667441595853,-21.8950109091289));
#78226=CARTESIAN_POINT('Ctrl Pts',(18.7090404529568,-21.0701050783104,-21.8906271574457));
#78227=CARTESIAN_POINT('Ctrl Pts',(18.7818648602089,-21.0697038545041,-21.8862434057626));
#78228=CARTESIAN_POINT('Ctrl Pts',(18.8543536318168,-21.0655761172261,-21.8818596540794));
#78229=CARTESIAN_POINT('Ctrl Pts',(18.896359511156,-21.063184171133,-21.8793193524552));
#78230=CARTESIAN_POINT('Ctrl Pts',(18.9382527891111,-21.0595418376991,-21.8767790508309));
#78231=CARTESIAN_POINT('Ctrl Pts',(18.979954172718,-21.054663916303,-21.8742387492067));
#78232=CARTESIAN_POINT('Ctrl Pts',(19.0521148572584,-21.0462230897252,-21.8698429740959));
#78233=CARTESIAN_POINT('Ctrl Pts',(19.1239758615628,-21.0340474581782,-21.8654471989851));
#78234=CARTESIAN_POINT('Ctrl Pts',(19.1951213386526,-21.0181694294126,-21.8610514238743));
#78235=CARTESIAN_POINT('Ctrl Pts',(19.2661639899332,-21.0023143489949,-21.856662001931));
#78236=CARTESIAN_POINT('Ctrl Pts',(19.3364927019385,-20.9827675991443,-21.8522725799877));
#78237=CARTESIAN_POINT('Ctrl Pts',(19.4056979906368,-20.959613212094,-21.8478831580444));
#78238=CARTESIAN_POINT('Ctrl Pts',(19.4748252628419,-20.936484927443,-21.8434986843834));
#78239=CARTESIAN_POINT('Ctrl Pts',(19.5428311742357,-20.9097572368777,-21.8391142107225));
#78240=CARTESIAN_POINT('Ctrl Pts',(19.6093192887935,-20.8795645625156,-21.8347297370615));
#78241=CARTESIAN_POINT('Ctrl Pts',(19.675767120119,-20.8493901810247,-21.8303479198267));
#78242=CARTESIAN_POINT('Ctrl Pts',(19.7406985429898,-20.8157551798471,-21.825966102592));
#78243=CARTESIAN_POINT('Ctrl Pts',(19.803736398282,-20.7788423681836,-21.8215842853572));
#78244=CARTESIAN_POINT('Ctrl Pts',(19.8667566475552,-20.7419398660025,-21.8172036919325));
#78245=CARTESIAN_POINT('Ctrl Pts',(19.9278839650038,-20.7017616137434,-21.8128230985077));
#78246=CARTESIAN_POINT('Ctrl Pts',(19.9867666083377,-20.6585359137838,-21.808442505083));
#78247=CARTESIAN_POINT('Ctrl Pts',(20.0456520352798,-20.6153081703798,-21.8040617045708));
#78248=CARTESIAN_POINT('Ctrl Pts',(20.1022921913093,-20.5690329791144,-21.7996809040586));
#78249=CARTESIAN_POINT('Ctrl Pts',(20.1563664498668,-20.519980447038,-21.7953001035464));
#78250=CARTESIAN_POINT('Ctrl Pts',(20.2104978279948,-20.4708760999272,-21.7909146755192));
#78251=CARTESIAN_POINT('Ctrl Pts',(20.2620575407503,-20.4189888782294,-21.786529247492));
#78252=CARTESIAN_POINT('Ctrl Pts',(20.3107606627202,-20.364626919076,-21.7821438194648));
#78253=CARTESIAN_POINT('Ctrl Pts',(20.3594910299654,-20.3102345490068,-21.7777559381617));
#78254=CARTESIAN_POINT('Ctrl Pts',(20.4053613227915,-20.2533650591673,-21.7733680568587));
#78255=CARTESIAN_POINT('Ctrl Pts',(20.4481276167033,-20.1943588505964,-21.7689801755556));
#78256=CARTESIAN_POINT('Ctrl Pts',(20.4909696471634,-20.1352481455596,-21.7645845235772));
#78257=CARTESIAN_POINT('Ctrl Pts',(20.5306964397318,-20.0739935686515,-21.7601888715988));
#78258=CARTESIAN_POINT('Ctrl Pts',(20.5671083269304,-20.0109631068826,-21.7557932196204));
#78259=CARTESIAN_POINT('Ctrl Pts',(20.5912144107273,-19.969234492684,-21.7528831272554));
#78260=CARTESIAN_POINT('Ctrl Pts',(20.613868534761,-19.9267280374392,-21.7499730348904));
#78261=CARTESIAN_POINT('Ctrl Pts',(20.6350243858782,-19.8835553039387,-21.7470629425253));
#78262=CARTESIAN_POINT('Ctrl Pts',(20.6668849852277,-19.8185373967291,-21.7426803588893));
#78263=CARTESIAN_POINT('Ctrl Pts',(20.6954698819653,-19.7517530160599,-21.7382977752533));
#78264=CARTESIAN_POINT('Ctrl Pts',(20.7205800139613,-19.6835660244499,-21.7339151916173));
#78265=CARTESIAN_POINT('Ctrl Pts',(20.7456523661794,-19.6154816244714,-21.7295392018549));
#78266=CARTESIAN_POINT('Ctrl Pts',(20.7672601652298,-19.5459992525245,-21.7251632120926));
#78267=CARTESIAN_POINT('Ctrl Pts',(20.7852510275153,-19.4755057039971,-21.7207872223302));
#78268=CARTESIAN_POINT('Ctrl Pts',(20.8032203357683,-19.4050966105787,-21.7164164752418));
#78269=CARTESIAN_POINT('Ctrl Pts',(20.8175811957868,-19.3336792133251,-21.7120457281534));
#78270=CARTESIAN_POINT('Ctrl Pts',(20.8282305507602,-19.2616569073388,-21.707674981065));
#78271=CARTESIAN_POINT('Ctrl Pts',(20.8388730093072,-19.1896812423493,-21.7033070644331));
#78272=CARTESIAN_POINT('Ctrl Pts',(20.845808660676,-19.1171019231659,-21.6989391478011));
#78273=CARTESIAN_POINT('Ctrl Pts',(20.8489855053725,-19.0443326164712,-21.6945712311692));
#78274=CARTESIAN_POINT('Ctrl Pts',(20.8521613481799,-18.9715862592065,-21.6902046920575));
#78275=CARTESIAN_POINT('Ctrl Pts',(20.8515807164049,-18.8986505164049,-21.6858381529459));
#78276=CARTESIAN_POINT('Ctrl Pts',(20.8472436019355,-18.8259425572265,-21.6814716138342));
#78277=CARTESIAN_POINT('Ctrl Pts',(20.8429064144311,-18.753233373679,-21.677105001192));
#78278=CARTESIAN_POINT('Ctrl Pts',(20.8348126494595,-18.6807524641984,-21.6727383885499));
#78279=CARTESIAN_POINT('Ctrl Pts',(20.8230143052733,-18.6089136663121,-21.6683717759077));
#78280=CARTESIAN_POINT('Ctrl Pts',(20.8112037490663,-18.5370005107965,-21.6640006435495));
#78281=CARTESIAN_POINT('Ctrl Pts',(20.7956810363731,-18.4657312722987,-21.6596295111913));
#78282=CARTESIAN_POINT('Ctrl Pts',(20.7765494969166,-18.3955105098514,-21.6552583788331));
#78283=CARTESIAN_POINT('Ctrl Pts',(20.7574075807255,-18.3252516604421,-21.6508848756213));
#78284=CARTESIAN_POINT('Ctrl Pts',(20.734653092167,-18.2560428791505,-21.6465113724094));
#78285=CARTESIAN_POINT('Ctrl Pts',(20.7084387230319,-18.1882718225755,-21.6421378691975));
#78286=CARTESIAN_POINT('Ctrl Pts',(20.6821776179286,-18.1203799411991,-21.6377565687388));
#78287=CARTESIAN_POINT('Ctrl Pts',(20.6524445121555,-18.0539313451297,-21.6333752682801));
#78288=CARTESIAN_POINT('Ctrl Pts',(20.619439293294,-17.9892914920377,-21.6289939678214));
#78289=CARTESIAN_POINT('Ctrl Pts',(20.5965714267485,-17.9445053768408,-21.6259583571622));
#78290=CARTESIAN_POINT('Ctrl Pts',(20.57213375941,-17.9005870397827,-21.622922746503));
#78291=CARTESIAN_POINT('Ctrl Pts',(20.546204814931,-17.8576496407728,-21.6198871358438));
#78292=CARTESIAN_POINT('Ctrl Pts',(20.5087128672688,-17.7955643245834,-21.6154977957359));
#78293=CARTESIAN_POINT('Ctrl Pts',(20.4679537715697,-17.7352871414802,-21.6111084556279));
#78294=CARTESIAN_POINT('Ctrl Pts',(20.4241273153556,-17.6771828923768,-21.60671911552));
#78295=CARTESIAN_POINT('Ctrl Pts',(20.3803658454572,-17.6191648008458,-21.6023362839703));
#78296=CARTESIAN_POINT('Ctrl Pts',(20.3335463321389,-17.5633136287167,-21.5979534524206));
#78297=CARTESIAN_POINT('Ctrl Pts',(20.283913029103,-17.5099671979401,-21.5935706208709));
#78298=CARTESIAN_POINT('Ctrl Pts',(20.2343380255226,-17.456683428072,-21.5891929374108));
#78299=CARTESIAN_POINT('Ctrl Pts',(20.1819561246821,-17.4058989062031,-21.5848152539507));
#78300=CARTESIAN_POINT('Ctrl Pts',(20.1270521542449,-17.3579188554049,-21.5804375704906));
#78301=CARTESIAN_POINT('Ctrl Pts',(20.0721829959018,-17.3099692265604,-21.5760626627192));
#78302=CARTESIAN_POINT('Ctrl Pts',(20.0147953030245,-17.2648208570169,-21.5716877549478));
#78303=CARTESIAN_POINT('Ctrl Pts',(19.9552100903752,-17.222741512912,-21.5673128471764));
#78304=CARTESIAN_POINT('Ctrl Pts',(19.8956430300011,-17.1806749880252,-21.5629392721942));
#78305=CARTESIAN_POINT('Ctrl Pts',(19.8338801725247,-17.1416759102888,-21.558565697212));
#78306=CARTESIAN_POINT('Ctrl Pts',(19.7702735413081,-17.1059701661173,-21.5541921222299));
#78307=CARTESIAN_POINT('Ctrl Pts',(19.7066653353733,-17.0702635379739,-21.5498184389705));
#78308=CARTESIAN_POINT('Ctrl Pts',(19.6412136864337,-17.0378506395157,-21.5454447557111));
#78309=CARTESIAN_POINT('Ctrl Pts',(19.5742959011684,-17.0089117882917,-21.5410710724518));
#78310=CARTESIAN_POINT('Ctrl Pts',(19.5073088887682,-16.9799429995295,-21.5366928645722));
#78311=CARTESIAN_POINT('Ctrl Pts',(19.4388531552012,-16.9544556253366,-21.5323146566927));
#78312=CARTESIAN_POINT('Ctrl Pts',(19.3693259376834,-16.9325817786039,-21.5279364488132));
#78313=CARTESIAN_POINT('Ctrl Pts',(19.2997608500006,-16.9106960175991,-21.5235558562063));
#78314=CARTESIAN_POINT('Ctrl Pts',(19.2291235834203,-16.8924278236772,-21.5191752635995));
#78315=CARTESIAN_POINT('Ctrl Pts',(19.1578238533414,-16.8778586496242,-21.5147946709926));
#78316=CARTESIAN_POINT('Ctrl Pts',(19.0863981311614,-16.8632637307212,-21.5104063375421));
#78317=CARTESIAN_POINT('Ctrl Pts',(19.0143080848955,-16.8523809568344,-21.5060180040915));
#78318=CARTESIAN_POINT('Ctrl Pts',(18.9419702886576,-16.8452400803519,-21.5016296706409));
#78319=CARTESIAN_POINT('Ctrl Pts',(18.8929666311248,-16.8404026497993,-21.4986568901481));
#78320=CARTESIAN_POINT('Ctrl Pts',(18.8438493706969,-16.8372813203535,-21.4956841096553));
#78321=CARTESIAN_POINT('Ctrl Pts',(18.7947475232676,-16.8358717575684,-21.4927113291624));
#78322=CARTESIAN_POINT('Ctrl Pts',(18.7222522474693,-16.8337906415164,-21.488322236837));
#78323=CARTESIAN_POINT('Ctrl Pts',(18.6495090698324,-16.8354351543627,-21.4839331445116));
#78324=CARTESIAN_POINT('Ctrl Pts',(18.5769328482517,-16.8408347033352,-21.4795440521862));
#78325=CARTESIAN_POINT('Ctrl Pts',(18.5044639925059,-16.8462262644699,-21.4751614528767));
#78326=CARTESIAN_POINT('Ctrl Pts',(18.4321620793838,-16.8553617985987,-21.4707788535672));
#78327=CARTESIAN_POINT('Ctrl Pts',(18.3604433407868,-16.868218720125,-21.4663962542577));
#78328=CARTESIAN_POINT('Ctrl Pts',(18.2888084465286,-16.8810606109898,-21.4620187785205));
#78329=CARTESIAN_POINT('Ctrl Pts',(18.2177558446894,-16.8976151620993,-21.4576413027833));
#78330=CARTESIAN_POINT('Ctrl Pts',(18.1476963106892,-16.917808026783,-21.4532638270461));
#78331=CARTESIAN_POINT('Ctrl Pts',(18.0776809567047,-16.9379881577097,-21.4488891117746));
#78332=CARTESIAN_POINT('Ctrl Pts',(18.0086578901714,-16.9618019166529,-21.4445143965032));
#78333=CARTESIAN_POINT('Ctrl Pts',(17.9410259673652,-16.9891242567175,-21.4401396812318));
#78334=CARTESIAN_POINT('Ctrl Pts',(17.8734144087345,-17.0164383699432,-21.4357662832003));
#78335=CARTESIAN_POINT('Ctrl Pts',(17.8071936089994,-17.0472587863894,-21.4313928851688));
#78336=CARTESIAN_POINT('Ctrl Pts',(17.7427439831315,-17.0814117211363,-21.4270194871373));
#78337=CARTESIAN_POINT('Ctrl Pts',(17.6782925274241,-17.1155656255459,-21.4226459649373));
#78338=CARTESIAN_POINT('Ctrl Pts',(17.6156127705188,-17.1530520085839,-21.4182724427373));
#78339=CARTESIAN_POINT('Ctrl Pts',(17.5550604851453,-17.1936511664877,-21.4138989205372));
#78340=CARTESIAN_POINT('Ctrl Pts',(17.4944451983904,-17.2342925656217,-21.4095208479236));
#78341=CARTESIAN_POINT('Ctrl Pts',(17.4359622039086,-17.2780529367419,-21.4051427753101));
#78342=CARTESIAN_POINT('Ctrl Pts',(17.3799375208464,-17.32466973157,-21.4007647026965));
#78343=CARTESIAN_POINT('Ctrl Pts',(17.3238821391245,-17.3713120700165,-21.3963842311231));
#78344=CARTESIAN_POINT('Ctrl Pts',(17.2702881051855,-17.4208136210669,-21.3920037595497));
#78345=CARTESIAN_POINT('Ctrl Pts',(17.2194455841251,-17.4728739332451,-21.3876232879764));
#78346=CARTESIAN_POINT('Ctrl Pts',(17.1685129338238,-17.5250265334594,-21.3832350510804));
#78347=CARTESIAN_POINT('Ctrl Pts',(17.120341855727,-17.5797465906982,-21.3788468141844));
#78348=CARTESIAN_POINT('Ctrl Pts',(17.0751827470182,-17.6366999121076,-21.3744585772885));
#78349=CARTESIAN_POINT('Ctrl Pts',(17.0445738554429,-17.6753029335072,-21.371484225686));
#78350=CARTESIAN_POINT('Ctrl Pts',(17.015347839445,-17.7149312818909,-21.3685098740835));
#78351=CARTESIAN_POINT('Ctrl Pts',(16.9875709599417,-17.7554739417626,-21.365535522481));
#78352=CARTESIAN_POINT('Ctrl Pts',(16.9460128347077,-17.8161314730044,-21.3610854734259));
#78353=CARTESIAN_POINT('Ctrl Pts',(16.9075410210167,-17.8790695324529,-21.3566354243708));
#78354=CARTESIAN_POINT('Ctrl Pts',(16.8724101016156,-17.9439464050791,-21.3521853753158));
#78355=CARTESIAN_POINT('Ctrl Pts',(16.8373354751619,-18.0087193205517,-21.3477424569132));
#78356=CARTESIAN_POINT('Ctrl Pts',(16.8055913305909,-18.0754244744595,-21.3432995385106));
#78357=CARTESIAN_POINT('Ctrl Pts',(16.77738933593,-18.1436908331291,-21.338856620108));
#78358=CARTESIAN_POINT('Ctrl Pts',(16.7492306468634,-18.2118523653399,-21.3344205240321));
#78359=CARTESIAN_POINT('Ctrl Pts',(16.7246034679416,-18.2815699082597,-21.3299844279563));
#78360=CARTESIAN_POINT('Ctrl Pts',(16.703673027533,-18.3524490139505,-21.3255483318804));
#78361=CARTESIAN_POINT('Ctrl Pts',(16.6827615762291,-18.4232638146991,-21.3211162604448));
#78362=CARTESIAN_POINT('Ctrl Pts',(16.6655403334367,-18.495237641409,-21.3166841890092));
#78363=CARTESIAN_POINT('Ctrl Pts',(16.6521256163152,-18.5679582697712,-21.3122521175736));
#78364=CARTESIAN_POINT('Ctrl Pts',(16.6387184414623,-18.6406380118066,-21.3078225380185));
#78365=CARTESIAN_POINT('Ctrl Pts',(16.6291136269053,-18.7140632656555,-21.3033929584635));
#78366=CARTESIAN_POINT('Ctrl Pts',(16.6233766956374,-18.7878102710847,-21.2989633789084));
#78367=CARTESIAN_POINT('Ctrl Pts',(16.6190996643447,-18.8427905794111,-21.2956610122798));
#78368=CARTESIAN_POINT('Ctrl Pts',(16.6169713926958,-18.8979494279291,-21.2923586456512));
#78369=CARTESIAN_POINT('Ctrl Pts',(16.6170002905213,-18.9531090839331,-21.2890562790225));
#78370=CARTESIAN_POINT('Ctrl Pts',(16.6170002427961,-18.9530139027121,-21.2873807947792));
#78371=CARTESIAN_POINT('Ctrl Pts',(16.6170353681744,-19.0263546841816,-21.283214403805));
#78372=CARTESIAN_POINT('Ctrl Pts',(16.620881643312,-19.099649181836,-21.2791526234396));
#78373=CARTESIAN_POINT('Ctrl Pts',(16.6454736247964,-19.3343610415228,-21.2662365927548));
#78374=CARTESIAN_POINT('Ctrl Pts',(16.6810044211168,-19.4936083875884,-21.257642580014));
#78375=CARTESIAN_POINT('Ctrl Pts',(16.7379955393082,-19.6575316163442,-21.2476766099661));
#78376=CARTESIAN_POINT('Ctrl Pts',(16.7416677446335,-19.6678357556093,-21.2470450721877));
#78377=CARTESIAN_POINT('Ctrl Pts',(16.745419449923,-19.6781104570625,-21.2464098137458));
#78378=CARTESIAN_POINT('Origin',(18.734,-18.952,0.));
#78379=CARTESIAN_POINT('',(16.7454193204094,-19.6781101023667,-20.4442392291799));
#78380=CARTESIAN_POINT('',(16.7454194499653,-19.6781104571783,-20.6683679347509));
#78381=CARTESIAN_POINT('',(16.7454194499637,-19.6781104571739,0.));
#78382=CARTESIAN_POINT('Ctrl Pts',(16.7454194499653,-19.6781104571783,-20.6683679347509));
#78383=CARTESIAN_POINT('Ctrl Pts',(16.7441348064984,-19.6745922362427,-20.668590378304));
#78384=CARTESIAN_POINT('Ctrl Pts',(16.7428594929539,-19.6710705874846,-20.6688125127429));
#78385=CARTESIAN_POINT('Ctrl Pts',(16.7369541278903,-19.6546273468838,-20.6698472702451));
#78386=CARTESIAN_POINT('Ctrl Pts',(16.7324404003774,-19.6416641112149,-20.6706560419502));
#78387=CARTESIAN_POINT('Ctrl Pts',(16.6991411812999,-19.5429488037885,-20.6767638054007));
#78388=CARTESIAN_POINT('Ctrl Pts',(16.6757501965837,-19.4554694899014,-20.6818794970702));
#78389=CARTESIAN_POINT('Ctrl Pts',(16.6306360858101,-19.2296586008703,-20.6946257394849));
#78390=CARTESIAN_POINT('Ctrl Pts',(16.6168948154608,-19.0901947037234,-20.7020607995078));
#78391=CARTESIAN_POINT('Ctrl Pts',(16.6170159593102,-18.9301096100918,-20.7109057137875));
#78392=CARTESIAN_POINT('Ctrl Pts',(16.6173229632374,-18.9098229033623,-20.7120327871212));
#78393=CARTESIAN_POINT('Ctrl Pts',(16.6196735652514,-18.830181690397,-20.7164920546507));
#78394=CARTESIAN_POINT('Ctrl Pts',(16.6239226589396,-18.7709248029925,-20.719885302315));
#78395=CARTESIAN_POINT('Ctrl Pts',(16.6316702790211,-18.7030447059488,-20.7239378573419));
#78396=CARTESIAN_POINT('Ctrl Pts',(16.6327408114508,-18.6941651491509,-20.7244712651555));
#78397=CARTESIAN_POINT('Ctrl Pts',(16.634438362504,-18.6807981222699,-20.7252795503377));
#78398=CARTESIAN_POINT('Ctrl Pts',(16.6350235902586,-18.6763053163335,-20.7255521289721));
#78399=CARTESIAN_POINT('Ctrl Pts',(16.636095341283,-18.6682787152921,-20.7260407764863));
#78400=CARTESIAN_POINT('Ctrl Pts',(16.6365763773781,-18.6647442403234,-20.7262565330954));
#78401=CARTESIAN_POINT('Ctrl Pts',(16.6376355527075,-18.6571063309708,-20.7267240521063));
#78402=CARTESIAN_POINT('Ctrl Pts',(16.6382167997036,-18.6530034304865,-20.7269759827503));
#78403=CARTESIAN_POINT('Ctrl Pts',(16.6398690487733,-18.6415821111098,-20.7276794391765));
#78404=CARTESIAN_POINT('Ctrl Pts',(16.6409663520168,-18.6342676419927,-20.7281324118739));
#78405=CARTESIAN_POINT('Ctrl Pts',(16.6474610426461,-18.5924691027289,-20.7307344389076));
#78406=CARTESIAN_POINT('Ctrl Pts',(16.6536719553288,-18.5581190719979,-20.7329253955482));
#78407=CARTESIAN_POINT('Ctrl Pts',(16.6761041931998,-18.4494703058947,-20.739990366585));
#78408=CARTESIAN_POINT('Ctrl Pts',(16.6954799886247,-18.3758873130994,-20.7449760055384));
#78409=CARTESIAN_POINT('Ctrl Pts',(16.7775784089416,-18.1207598411494,-20.7626582096691));
#78410=CARTESIAN_POINT('Ctrl Pts',(16.8609882798593,-17.9468118002398,-20.7753361225597));
#78411=CARTESIAN_POINT('Ctrl Pts',(16.9785112585037,-17.7686123322985,-20.7884543812594));
#78412=CARTESIAN_POINT('Ctrl Pts',(16.9905654135348,-17.7509242367354,-20.7897596025357));
#78413=CARTESIAN_POINT('Ctrl Pts',(17.0076899876059,-17.7265970495096,-20.7915596575448));
#78414=CARTESIAN_POINT('Ctrl Pts',(17.0125342438745,-17.7198010292286,-20.7920630665967));
#78415=CARTESIAN_POINT('Ctrl Pts',(17.020958416024,-17.7081293818748,-20.7929286403344));
#78416=CARTESIAN_POINT('Ctrl Pts',(17.024519245586,-17.7032401613862,-20.793291534835));
#78417=CARTESIAN_POINT('Ctrl Pts',(17.0319299155845,-17.6931559926561,-20.7940406860232));
#78418=CARTESIAN_POINT('Ctrl Pts',(17.0357827044739,-17.6879632815084,-20.7944268228754));
#78419=CARTESIAN_POINT('Ctrl Pts',(17.0448502384326,-17.6758585304046,-20.7953278661294));
#78420=CARTESIAN_POINT('Ctrl Pts',(17.0500837422373,-17.6689606367444,-20.7958420316204));
#78421=CARTESIAN_POINT('Ctrl Pts',(17.0671665414274,-17.6467296366344,-20.7975015884365));
#78422=CARTESIAN_POINT('Ctrl Pts',(17.0791842933618,-17.6315267840458,-20.7986403172642));
#78423=CARTESIAN_POINT('Ctrl Pts',(17.1414401067977,-17.5549561348447,-20.8043989609493));
#78424=CARTESIAN_POINT('Ctrl Pts',(17.1948920696731,-17.4962777335467,-20.8088862716222));
#78425=CARTESIAN_POINT('Ctrl Pts',(17.3679310293639,-17.3265344580812,-20.8223348122778));
#78426=CARTESIAN_POINT('Ctrl Pts',(17.4971413356927,-17.2261791559357,-20.8309358352439));
#78427=CARTESIAN_POINT('Ctrl Pts',(17.6888224651241,-17.1099834120811,-20.8434650927113));
#78428=CARTESIAN_POINT('Ctrl Pts',(17.7424062160291,-17.0805937133456,-20.8469515463375));
#78429=CARTESIAN_POINT('Ctrl Pts',(17.8053528508124,-17.0495314623582,-20.8511147112887));
#78430=CARTESIAN_POINT('Ctrl Pts',(17.8135516627711,-17.0455512290744,-20.8516582496761));
#78431=CARTESIAN_POINT('Ctrl Pts',(17.8258413198441,-17.0396827906079,-20.8524752803578));
#78432=CARTESIAN_POINT('Ctrl Pts',(17.829913030924,-17.0377544438696,-20.8527463458961));
#78433=CARTESIAN_POINT('Ctrl Pts',(17.837219177645,-17.0343227909233,-20.8532334596924));
#78434=CARTESIAN_POINT('Ctrl Pts',(17.8404512827568,-17.0328146490828,-20.8534492048724));
#78435=CARTESIAN_POINT('Ctrl Pts',(17.8474674131497,-17.0295623982225,-20.8539181004368));
#78436=CARTESIAN_POINT('Ctrl Pts',(17.8512527308801,-17.027821313275,-20.8541714267524));
#78437=CARTESIAN_POINT('Ctrl Pts',(17.8618590201682,-17.0229807559241,-20.8548821606054));
#78438=CARTESIAN_POINT('Ctrl Pts',(17.8686912632587,-17.0199063379374,-20.8553410607026));
#78439=CARTESIAN_POINT('Ctrl Pts',(17.9088201517114,-17.0021044161471,-20.8580420077365));
#78440=CARTESIAN_POINT('Ctrl Pts',(17.9424738266147,-16.9882025261106,-20.8603296450267));
#78441=CARTESIAN_POINT('Ctrl Pts',(18.0526121619314,-16.9459967134346,-20.8678505797909));
#78442=CARTESIAN_POINT('Ctrl Pts',(18.1303751010118,-16.9212430486737,-20.8732107040317));
#78443=CARTESIAN_POINT('Ctrl Pts',(18.3869084934598,-16.8556220732748,-20.8906947769685));
#78444=CARTESIAN_POINT('Ctrl Pts',(18.5696370356424,-16.8334428624919,-20.9027594149921));
#78445=CARTESIAN_POINT('Ctrl Pts',(18.7752757176076,-16.8352847894356,-20.9154088510647));
#78446=CARTESIAN_POINT('Ctrl Pts',(18.7975860889257,-16.8358374739657,-20.9167705181314));
#78447=CARTESIAN_POINT('Ctrl Pts',(18.828370448187,-16.8370873888204,-20.9186352166078));
#78448=CARTESIAN_POINT('Ctrl Pts',(18.8368545988943,-16.8374830175211,-20.9191476427989));
#78449=CARTESIAN_POINT('Ctrl Pts',(18.8514163840271,-16.8382499051485,-20.920024659769));
#78450=CARTESIAN_POINT('Ctrl Pts',(18.8574951702196,-16.8385963436061,-20.9203900242773));
#78451=CARTESIAN_POINT('Ctrl Pts',(18.8700077345155,-16.8393636221401,-20.9211405879507));
#78452=CARTESIAN_POINT('Ctrl Pts',(18.876441259797,-16.8397876390306,-20.921525683414));
#78453=CARTESIAN_POINT('Ctrl Pts',(18.8913807799879,-16.8408408313187,-20.9224180718585));
#78454=CARTESIAN_POINT('Ctrl Pts',(18.8998851476281,-16.8414920359164,-20.9229246681711));
#78455=CARTESIAN_POINT('Ctrl Pts',(18.926981877434,-16.8437317094449,-20.9245344936403));
#78456=CARTESIAN_POINT('Ctrl Pts',(18.9455575972416,-16.8455146318989,-20.9256316173553));
#78457=CARTESIAN_POINT('Ctrl Pts',(19.1238293861668,-16.8650074144962,-20.936104584212));
#78458=CARTESIAN_POINT('Ctrl Pts',(19.2810467987769,-16.9005973171631,-20.944851943207));
#78459=CARTESIAN_POINT('Ctrl Pts',(19.5595112982897,-16.9979642147191,-20.9608716902572));
#78460=CARTESIAN_POINT('Ctrl Pts',(19.6817599775027,-17.0542471539759,-20.9681342243965));
#78461=CARTESIAN_POINT('Ctrl Pts',(19.8113925966665,-17.1295949860951,-20.9769255599056));
#78462=CARTESIAN_POINT('Ctrl Pts',(19.8248600163339,-17.1376242852256,-20.9778530720793));
#78463=CARTESIAN_POINT('Ctrl Pts',(19.843175667546,-17.1488217361748,-20.9791357894353));
#78464=CARTESIAN_POINT('Ctrl Pts',(19.8481023036346,-17.1518615142572,-20.9794829568611));
#78465=CARTESIAN_POINT('Ctrl Pts',(19.8559119558499,-17.1567244782742,-20.9800367880161));
#78466=CARTESIAN_POINT('Ctrl Pts',(19.858803181974,-17.1585345174698,-20.9802425906215));
#78467=CARTESIAN_POINT('Ctrl Pts',(19.8647630702242,-17.1622857591029,-20.9806684406013));
#78468=CARTESIAN_POINT('Ctrl Pts',(19.8678311048603,-17.1642278640955,-20.9808885509505));
#78469=CARTESIAN_POINT('Ctrl Pts',(19.8751297553507,-17.1688743472511,-20.9814142824791));
#78470=CARTESIAN_POINT('Ctrl Pts',(19.8793557607971,-17.1715858930986,-20.9817203767317));
#78471=CARTESIAN_POINT('Ctrl Pts',(19.8935799345559,-17.1807841979277,-20.9827562531188));
#78472=CARTESIAN_POINT('Ctrl Pts',(19.9035327475494,-17.1873402085578,-20.9834904469937));
#78473=CARTESIAN_POINT('Ctrl Pts',(19.9273112382603,-17.20329284101,-20.9852661632181));
#78474=CARTESIAN_POINT('Ctrl Pts',(19.9410818220879,-17.2127697457847,-20.9863123317198));
#78475=CARTESIAN_POINT('Ctrl Pts',(19.9923064800113,-17.248923887959,-20.9902670048094));
#78476=CARTESIAN_POINT('Ctrl Pts',(20.0289984831854,-17.2766547150036,-20.9932278203942));
#78477=CARTESIAN_POINT('Ctrl Pts',(20.1225696448146,-17.3522846175853,-21.0010639595944));
#78478=CARTESIAN_POINT('Ctrl Pts',(20.17788036306,-17.4020245455899,-21.0059870821838));
#78479=CARTESIAN_POINT('Ctrl Pts',(20.340265877829,-17.564304632727,-21.0211539576285));
#78480=CARTESIAN_POINT('Ctrl Pts',(20.4376882469793,-17.6858043470796,-21.031270219651));
#78481=CARTESIAN_POINT('Ctrl Pts',(20.5337906378363,-17.8370938509968,-21.0423125609111));
#78482=CARTESIAN_POINT('Ctrl Pts',(20.5462830395389,-17.8575173278558,-21.0437748160134));
#78483=CARTESIAN_POINT('Ctrl Pts',(20.5633463525542,-17.8865071637873,-21.0458116441825));
#78484=CARTESIAN_POINT('Ctrl Pts',(20.5682085162694,-17.894899160264,-21.0463967903385));
#78485=CARTESIAN_POINT('Ctrl Pts',(20.5759804390449,-17.9085284141976,-21.0473399870257));
#78486=CARTESIAN_POINT('Ctrl Pts',(20.5789258966666,-17.9137450577254,-21.047699324951));
#78487=CARTESIAN_POINT('Ctrl Pts',(20.585018155475,-17.9246427286944,-21.048446539027));
#78488=CARTESIAN_POINT('Ctrl Pts',(20.5881610425254,-17.9303258813913,-21.0488342716484));
#78489=CARTESIAN_POINT('Ctrl Pts',(20.5955279171313,-17.9437930548324,-21.0497485408661));
#78490=CARTESIAN_POINT('Ctrl Pts',(20.5997293309015,-17.9515893353267,-21.0502742671338));
#78491=CARTESIAN_POINT('Ctrl Pts',(20.6135045226626,-17.9775396546421,-21.0520126166771));
#78492=CARTESIAN_POINT('Ctrl Pts',(20.6228634135764,-17.9958068898118,-21.0532176350391));
#78493=CARTESIAN_POINT('Ctrl Pts',(20.6710804835961,-18.0933912503387,-21.0595612182483));
#78494=CARTESIAN_POINT('Ctrl Pts',(20.705214392142,-18.1749503421696,-21.0645333127584));
#78495=CARTESIAN_POINT('Ctrl Pts',(20.7770394327539,-18.3820778355627,-21.0766340371412));
#78496=CARTESIAN_POINT('Ctrl Pts',(20.8083599893668,-18.5094499401615,-21.0836114699341));
#78497=CARTESIAN_POINT('Ctrl Pts',(20.833296192086,-18.6761974614834,-21.0929116951813));
#78498=CARTESIAN_POINT('Ctrl Pts',(20.8378764044661,-18.713640216961,-21.0950120356838));
#78499=CARTESIAN_POINT('Ctrl Pts',(20.8458049312631,-18.7968456367883,-21.0997433823018));
#78500=CARTESIAN_POINT('Ctrl Pts',(20.8486704702366,-18.842633321617,-21.1023896304583));
#78501=CARTESIAN_POINT('Ctrl Pts',(20.8502755294736,-18.8960977918028,-21.1055661138367));
#78502=CARTESIAN_POINT('Ctrl Pts',(20.8504631957338,-18.9037225656617,-21.1060211766074));
#78503=CARTESIAN_POINT('Ctrl Pts',(20.8506981199302,-18.9159542766341,-21.1067547192797));
#78504=CARTESIAN_POINT('Ctrl Pts',(20.8507715502729,-18.9205607232214,-21.1070317729793));
#78505=CARTESIAN_POINT('Ctrl Pts',(20.8508753357168,-18.9287483570312,-21.1075257003794));
#78506=CARTESIAN_POINT('Ctrl Pts',(20.8509116405735,-18.9323294209292,-21.1077422381226));
#78507=CARTESIAN_POINT('Ctrl Pts',(20.8509695834459,-18.9399531742319,-21.1082043236871));
#78508=CARTESIAN_POINT('Ctrl Pts',(20.8509887281269,-18.9439957762768,-21.1084500024256));
#78509=CARTESIAN_POINT('Ctrl Pts',(20.8510092759738,-18.9549760307021,-21.1091190226478));
#78510=CARTESIAN_POINT('Ctrl Pts',(20.8509881550678,-18.9619136038538,-21.1095435935371));
#78511=CARTESIAN_POINT('Ctrl Pts',(20.8507067513094,-18.9972657303104,-21.1117161927685));
#78512=CARTESIAN_POINT('Ctrl Pts',(20.8499084969048,-19.0256716116516,-21.1134918173908));
#78513=CARTESIAN_POINT('Ctrl Pts',(20.8458833591939,-19.1090740112288,-21.1187766106147));
#78514=CARTESIAN_POINT('Ctrl Pts',(20.841081398104,-19.1639686715603,-21.1223459901169));
#78515=CARTESIAN_POINT('Ctrl Pts',(20.8165236137624,-19.3574160321671,-21.1351168642238));
#78516=CARTESIAN_POINT('Ctrl Pts',(20.7851821639716,-19.4941470826533,-21.1444681992938));
#78517=CARTESIAN_POINT('Ctrl Pts',(20.7117607576932,-19.7124765734288,-21.1593417742929));
#78518=CARTESIAN_POINT('Ctrl Pts',(20.6774820193082,-19.7962414439341,-21.1650403526591));
#78519=CARTESIAN_POINT('Ctrl Pts',(20.6319427774607,-19.8899183348006,-21.1713958232838));
#78520=CARTESIAN_POINT('Ctrl Pts',(20.625818564718,-19.9022105668768,-21.1722295668832));
#78521=CARTESIAN_POINT('Ctrl Pts',(20.6158042833255,-19.9218301055949,-21.1735601516639));
#78522=CARTESIAN_POINT('Ctrl Pts',(20.6119900834166,-19.9291954994298,-21.1740596352053));
#78523=CARTESIAN_POINT('Ctrl Pts',(20.6051403519625,-19.9422344075863,-21.1749438714527));
#78524=CARTESIAN_POINT('Ctrl Pts',(20.602122073986,-19.9479168222362,-21.1753292269818));
#78525=CARTESIAN_POINT('Ctrl Pts',(20.5957788408268,-19.9597287192617,-21.1761302977887));
#78526=CARTESIAN_POINT('Ctrl Pts',(20.5924494089736,-19.9658557194433,-21.1765458481905));
#78527=CARTESIAN_POINT('Ctrl Pts',(20.5837231444416,-19.9817268370587,-21.1776224012723));
#78528=CARTESIAN_POINT('Ctrl Pts',(20.578279529071,-19.9914450903525,-21.1782817260884));
#78529=CARTESIAN_POINT('Ctrl Pts',(20.5542939886397,-20.0334837843617,-21.1811348734192));
#78530=CARTESIAN_POINT('Ctrl Pts',(20.5349766166401,-20.0653556740046,-21.1833006274091));
#78531=CARTESIAN_POINT('Ctrl Pts',(20.4814022596282,-20.1487019246783,-21.1889868978582));
#78532=CARTESIAN_POINT('Ctrl Pts',(20.4457144124919,-20.1992148099006,-21.1924562679554));
#78533=CARTESIAN_POINT('Ctrl Pts',(20.3212188357911,-20.3599966382228,-21.203706746279));
#78534=CARTESIAN_POINT('Ctrl Pts',(20.2235750955592,-20.4629208706177,-21.2112292798062));
#78535=CARTESIAN_POINT('Ctrl Pts',(20.0589846054194,-20.6048312739061,-21.2232594631871));
#78536=CARTESIAN_POINT('Ctrl Pts',(19.9989617028074,-20.6512070870442,-21.2275423201506));
#78537=CARTESIAN_POINT('Ctrl Pts',(19.9287634567381,-20.6996612096779,-21.232597429934));
#78538=CARTESIAN_POINT('Ctrl Pts',(19.9209015376318,-20.7050100267027,-21.2331642151306));
#78539=CARTESIAN_POINT('Ctrl Pts',(19.9091942263251,-20.7128601792525,-21.2340095820793));
#78540=CARTESIAN_POINT('Ctrl Pts',(19.9053761836469,-20.715402357927,-21.2342854892835));
#78541=CARTESIAN_POINT('Ctrl Pts',(19.8985629713055,-20.7199069285266,-21.2347782736967));
#78542=CARTESIAN_POINT('Ctrl Pts',(19.8955710575026,-20.7218741481059,-21.2349948230819));
#78543=CARTESIAN_POINT('Ctrl Pts',(19.8891185625986,-20.7260933326153,-21.2354621790106));
#78544=CARTESIAN_POINT('Ctrl Pts',(19.8856564244501,-20.7283427388438,-21.2357131445364));
#78545=CARTESIAN_POINT('Ctrl Pts',(19.8760732416528,-20.734529292701,-21.2364083233809));
#78546=CARTESIAN_POINT('Ctrl Pts',(19.8699385072232,-20.7384449817777,-21.236853916029));
#78547=CARTESIAN_POINT('Ctrl Pts',(19.8360663291079,-20.759819958445,-21.239316789699));
#78548=CARTESIAN_POINT('Ctrl Pts',(19.8079481125203,-20.7766639072493,-21.2413707537187));
#78549=CARTESIAN_POINT('Ctrl Pts',(19.637133811473,-20.8736725923874,-21.253852858953));
#78550=CARTESIAN_POINT('Ctrl Pts',(19.4859266550713,-20.9377197301571,-21.2648703773371));
#78551=CARTESIAN_POINT('Ctrl Pts',(19.219052034435,-21.0158563298912,-21.2830111543928));
#78552=CARTESIAN_POINT('Ctrl Pts',(19.1068139143064,-21.0390542714415,-21.2902909846396));
#78553=CARTESIAN_POINT('Ctrl Pts',(18.9790747482339,-21.0548149962688,-21.2981493777544));
#78554=CARTESIAN_POINT('Ctrl Pts',(18.9648977846834,-21.0564188673792,-21.2990159480795));
#78555=CARTESIAN_POINT('Ctrl Pts',(18.9422913718601,-21.0587451792277,-21.3003891073552));
#78556=CARTESIAN_POINT('Ctrl Pts',(18.933872123076,-21.0595606001829,-21.3008986009188));
#78557=CARTESIAN_POINT('Ctrl Pts',(18.9190045968664,-21.0609106572923,-21.301795011777));
#78558=CARTESIAN_POINT('Ctrl Pts',(18.9125583738391,-21.0614662286638,-21.3021825812551));
#78559=CARTESIAN_POINT('Ctrl Pts',(18.8992101478361,-21.0625550281615,-21.3029828981746));
#78560=CARTESIAN_POINT('Ctrl Pts',(18.8923078657119,-21.0630839730446,-21.3033955068471));
#78561=CARTESIAN_POINT('Ctrl Pts',(18.8745625674112,-21.0643563347267,-21.3044532004385));
#78562=CARTESIAN_POINT('Ctrl Pts',(18.8637161113918,-21.0650501312834,-21.3050967260024));
#78563=CARTESIAN_POINT('Ctrl Pts',(18.8182383210541,-21.0676076382278,-21.307782974265));
#78564=CARTESIAN_POINT('Ctrl Pts',(18.7835680456845,-21.0687038019414,-21.3098016620234));
#78565=CARTESIAN_POINT('Ctrl Pts',(18.6930029358653,-21.0693405949672,-21.3150107968876));
#78566=CARTESIAN_POINT('Ctrl Pts',(18.637124726158,-21.0675206934193,-21.3181606462064));
#78567=CARTESIAN_POINT('Ctrl Pts',(18.3834490253179,-21.0491849388313,-21.3322947223814));
#78568=CARTESIAN_POINT('Ctrl Pts',(18.1885432697126,-21.007122439283,-21.3426052567678));
#78569=CARTESIAN_POINT('Ctrl Pts',(17.9724265963165,-20.9275285600448,-21.3558294338989));
#78570=CARTESIAN_POINT('Ctrl Pts',(17.9427393213528,-20.9158262226672,-21.3576899849543));
#78571=CARTESIAN_POINT('Ctrl Pts',(17.9070443376312,-20.9008149796076,-21.3599939051993));
#78572=CARTESIAN_POINT('Ctrl Pts',(17.9007719012643,-20.8981414195499,-21.3604012976031));
#78573=CARTESIAN_POINT('Ctrl Pts',(17.8904606766489,-20.8936873824995,-21.3610753741911));
#78574=CARTESIAN_POINT('Ctrl Pts',(17.8864142923849,-20.8919244698782,-21.3613410118751));
#78575=CARTESIAN_POINT('Ctrl Pts',(17.8791233500635,-20.8887208152821,-21.3618217113354));
#78576=CARTESIAN_POINT('Ctrl Pts',(17.8758768732385,-20.8872845532682,-21.362036496941));
#78577=CARTESIAN_POINT('Ctrl Pts',(17.8695652741977,-20.8844732572644,-21.3624555348091));
#78578=CARTESIAN_POINT('Ctrl Pts',(17.8664998554812,-20.8830991129689,-21.3626597245703));
#78579=CARTESIAN_POINT('Ctrl Pts',(17.8574561994662,-20.8790192075954,-21.3632640852242));
#78580=CARTESIAN_POINT('Ctrl Pts',(17.8514873236632,-20.8762929699415,-21.3636654975209));
#78581=CARTESIAN_POINT('Ctrl Pts',(17.8231312490501,-20.8631818732934,-21.3655841969521));
#78582=CARTESIAN_POINT('Ctrl Pts',(17.8009151237192,-20.8524342987479,-21.3671223449005));
#78583=CARTESIAN_POINT('Ctrl Pts',(17.7387161835997,-20.8209905937864,-21.3715175782383));
#78584=CARTESIAN_POINT('Ctrl Pts',(17.6991998507323,-20.7994046232302,-21.3744154243017));
#78585=CARTESIAN_POINT('Ctrl Pts',(17.5784756444411,-20.7283695383323,-21.3835372013532));
#78586=CARTESIAN_POINT('Ctrl Pts',(17.4998886812953,-20.6746996142006,-21.3898623194032));
#78587=CARTESIAN_POINT('Ctrl Pts',(17.3073656436015,-20.523263804994,-21.4060185095361));
#78588=CARTESIAN_POINT('Ctrl Pts',(17.1997104958011,-20.4183312382949,-21.4156928955309));
#78589=CARTESIAN_POINT('Ctrl Pts',(17.095014197546,-20.2920052958014,-21.4257089375579));
#78590=CARTESIAN_POINT('Ctrl Pts',(17.0861067224719,-20.2810358966566,-21.4265670572121));
#78591=CARTESIAN_POINT('Ctrl Pts',(17.0720934640097,-20.2634213138756,-21.4279268883053));
#78592=CARTESIAN_POINT('Ctrl Pts',(17.0669162730053,-20.2568337239732,-21.4284314759978));
#78593=CARTESIAN_POINT('Ctrl Pts',(17.0578483390237,-20.2451533856107,-21.4293192434309));
#78594=CARTESIAN_POINT('Ctrl Pts',(17.0539413835426,-20.2400734124992,-21.4297030690241));
#78595=CARTESIAN_POINT('Ctrl Pts',(17.045902570356,-20.2295222394312,-21.4304956168759));
#78596=CARTESIAN_POINT('Ctrl Pts',(17.041774097975,-20.2240485456295,-21.4309042020828));
#78597=CARTESIAN_POINT('Ctrl Pts',(17.0312338007196,-20.2099316687941,-21.4319514451176));
#78598=CARTESIAN_POINT('Ctrl Pts',(17.0248611085845,-20.2012594082619,-21.4325885617407));
#78599=CARTESIAN_POINT('Ctrl Pts',(16.998453023494,-20.1647417077541,-21.4352459079932));
#78600=CARTESIAN_POINT('Ctrl Pts',(16.9790291445457,-20.1364590544198,-21.4372424437986));
#78601=CARTESIAN_POINT('Ctrl Pts',(16.9301557786891,-20.0614521293199,-21.4423912249897));
#78602=CARTESIAN_POINT('Ctrl Pts',(16.9018314005475,-20.0140248948994,-21.4455035981185));
#78603=CARTESIAN_POINT('Ctrl Pts',(16.8405504664467,-19.9016494245699,-21.4526165630114));
#78604=CARTESIAN_POINT('Ctrl Pts',(16.809025281103,-19.8360012188719,-21.4565793344688));
#78605=CARTESIAN_POINT('Ctrl Pts',(16.7684068302387,-19.7388850155352,-21.4622948397039));
#78606=CARTESIAN_POINT('Ctrl Pts',(16.7565625548255,-19.7086277997814,-21.4640561247131));
#78607=CARTESIAN_POINT('Ctrl Pts',(16.7454194499919,-19.678110457251,-21.4658225324418));
#78608=CARTESIAN_POINT('Ctrl Pts',(16.745419449923,-19.6781104570625,-21.2464098137458));
#78609=CARTESIAN_POINT('Ctrl Pts',(16.7527636255383,-19.6982237671557,-21.2451662593623));
#78610=CARTESIAN_POINT('Ctrl Pts',(16.7604124473736,-19.7182242707579,-21.2439084485296));
#78611=CARTESIAN_POINT('Ctrl Pts',(16.7710457043463,-19.7448124735101,-21.2422034349802));
#78612=CARTESIAN_POINT('Ctrl Pts',(16.7737624299642,-19.7515060040884,-21.241771382987));
#78613=CARTESIAN_POINT('Ctrl Pts',(16.7780760232234,-19.7619797753612,-21.241090700836));
#78614=CARTESIAN_POINT('Ctrl Pts',(16.7796497446164,-19.7657695730657,-21.2408434511686));
#78615=CARTESIAN_POINT('Ctrl Pts',(16.7826135719917,-19.7728488054705,-21.2403797672208));
#78616=CARTESIAN_POINT('Ctrl Pts',(16.7840009862905,-19.7761393078273,-21.2401634966048));
#78617=CARTESIAN_POINT('Ctrl Pts',(16.7871885268885,-19.7836460214901,-21.2396684192655));
#78618=CARTESIAN_POINT('Ctrl Pts',(16.7889940230661,-19.7878598959617,-21.2393892888697));
#78619=CARTESIAN_POINT('Ctrl Pts',(16.7945883559339,-19.8008003200464,-21.2385284233604));
#78620=CARTESIAN_POINT('Ctrl Pts',(16.798422280582,-19.809507080309,-21.2379440407997));
#78621=CARTESIAN_POINT('Ctrl Pts',(16.851424787907,-19.927708005361,-21.2299430499284));
#78622=CARTESIAN_POINT('Ctrl Pts',(16.9097546367613,-20.0328412114739,-21.222046249565));
#78623=CARTESIAN_POINT('Ctrl Pts',(17.0373577043262,-20.2228030219735,-21.2069280582549));
#78624=CARTESIAN_POINT('Ctrl Pts',(17.1049303948756,-20.3083447574048,-21.1997344815819));
#78625=CARTESIAN_POINT('Ctrl Pts',(17.2157356654224,-20.4283225590371,-21.1892424346618));
#78626=CARTESIAN_POINT('Ctrl Pts',(17.2542172143822,-20.4668922699957,-21.1857953784389));
#78627=CARTESIAN_POINT('Ctrl Pts',(17.310715173096,-20.5193098408933,-21.1810061335353));
#78628=CARTESIAN_POINT('Ctrl Pts',(17.327529678,-20.5344162318493,-21.1796125375574));
#78629=CARTESIAN_POINT('Ctrl Pts',(17.3536852690417,-20.5571684568501,-21.1774922913361));
#78630=CARTESIAN_POINT('Ctrl Pts',(17.3628547924315,-20.5650081712708,-21.1767576852892));
#78631=CARTESIAN_POINT('Ctrl Pts',(17.3799883106688,-20.579405219871,-21.1754009323345));
#78632=CARTESIAN_POINT('Ctrl Pts',(17.3879341446112,-20.5859835137969,-21.1747779378894));
#78633=CARTESIAN_POINT('Ctrl Pts',(17.401101328972,-20.5967232909328,-21.1737556316717));
#78634=CARTESIAN_POINT('Ctrl Pts',(17.40629478113,-20.6009185620697,-21.1733549545101));
#78635=CARTESIAN_POINT('Ctrl Pts',(17.4165517911981,-20.6091242977851,-21.1725685706118));
#78636=CARTESIAN_POINT('Ctrl Pts',(17.4216140267495,-20.6131362917674,-21.1721828049434));
#78637=CARTESIAN_POINT('Ctrl Pts',(17.4333466046785,-20.6223476493514,-21.1712940795849));
#78638=CARTESIAN_POINT('Ctrl Pts',(17.4400299285359,-20.6275303583568,-21.1707917859344));
#78639=CARTESIAN_POINT('Ctrl Pts',(17.4580911914217,-20.6413637847229,-21.1694448336001));
#78640=CARTESIAN_POINT('Ctrl Pts',(17.4695261004689,-20.6499396506526,-21.1686031158945));
#78641=CARTESIAN_POINT('Ctrl Pts',(17.5749932258708,-20.7273806910733,-21.160937700305));
#78642=CARTESIAN_POINT('Ctrl Pts',(17.6744809196387,-20.7884906340283,-21.1544288556416));
#78643=CARTESIAN_POINT('Ctrl Pts',(17.924069777241,-20.9147306291121,-21.1391142841543));
#78644=CARTESIAN_POINT('Ctrl Pts',(18.0776371463879,-20.9712756947479,-21.1304943329389));
#78645=CARTESIAN_POINT('Ctrl Pts',(18.2675045627371,-21.0172146651587,-21.1192744585072));
#78646=CARTESIAN_POINT('Ctrl Pts',(18.2990256928423,-21.0240826969062,-21.1173926007298));
#78647=CARTESIAN_POINT('Ctrl Pts',(18.3377825562967,-21.0316040355389,-21.1150418377291));
#78648=CARTESIAN_POINT('Ctrl Pts',(18.3448825713782,-21.0329442161303,-21.1146096851959));
#78649=CARTESIAN_POINT('Ctrl Pts',(18.3560299249902,-21.0349893181378,-21.1139286267818));
#78650=CARTESIAN_POINT('Ctrl Pts',(18.3600727685966,-21.035718863483,-21.1136810984186));
#78651=CARTESIAN_POINT('Ctrl Pts',(18.3676364747793,-21.0370610396962,-21.1132169728438));
#78652=CARTESIAN_POINT('Ctrl Pts',(18.371156773337,-21.0376765243169,-21.1130005399103));
#78653=CARTESIAN_POINT('Ctrl Pts',(18.3792007882109,-21.0390619483075,-21.1125050327027));
#78654=CARTESIAN_POINT('Ctrl Pts',(18.3837254427443,-21.0398260919873,-21.1122256346616));
#78655=CARTESIAN_POINT('Ctrl Pts',(18.3955457486324,-21.0417828521001,-21.1114940145469));
#78656=CARTESIAN_POINT('Ctrl Pts',(18.4028451529991,-21.0429519633025,-21.111040513112));
#78657=CARTESIAN_POINT('Ctrl Pts',(18.4508057912219,-21.0503761594953,-21.1080502836029));
#78658=CARTESIAN_POINT('Ctrl Pts',(18.4916330076758,-21.0554826346607,-21.1054554074111));
#78659=CARTESIAN_POINT('Ctrl Pts',(18.6965047503879,-21.0750638190948,-21.0922721036984));
#78660=CARTESIAN_POINT('Ctrl Pts',(18.8616967296209,-21.0715523984599,-21.0811771138372));
#78661=CARTESIAN_POINT('Ctrl Pts',(19.1200097550326,-21.0357277959425,-21.0642237547855));
#78662=CARTESIAN_POINT('Ctrl Pts',(19.214203247993,-21.0160577126116,-21.0581157048154));
#78663=CARTESIAN_POINT('Ctrl Pts',(19.3274215847616,-20.9842404114641,-21.0508911665999));
#78664=CARTESIAN_POINT('Ctrl Pts',(19.3480087226243,-20.9781153987704,-21.0495819749366));
#78665=CARTESIAN_POINT('Ctrl Pts',(19.3771092351514,-20.9689732153594,-21.0477371963725));
#78666=CARTESIAN_POINT('Ctrl Pts',(19.3857014885393,-20.9662133982257,-21.0471932264209));
#78667=CARTESIAN_POINT('Ctrl Pts',(19.4004794163168,-20.9613622912994,-21.0462588160613));
#78668=CARTESIAN_POINT('Ctrl Pts',(19.4066734945251,-20.9592971880905,-21.0458675197625));
#78669=CARTESIAN_POINT('Ctrl Pts',(19.418505085799,-20.9552916244121,-21.0451207326991));
#78670=CARTESIAN_POINT('Ctrl Pts',(19.4241441400081,-20.9533559433685,-21.0447650884325));
#78671=CARTESIAN_POINT('Ctrl Pts',(19.4387648011857,-20.9482680628082,-21.04384368301));
#78672=CARTESIAN_POINT('Ctrl Pts',(19.4477335235512,-20.9450790414422,-21.0432791473921));
#78673=CARTESIAN_POINT('Ctrl Pts',(19.4781319616414,-20.9340387192806,-21.0413677901164));
#78674=CARTESIAN_POINT('Ctrl Pts',(19.4994565717454,-20.925901253218,-21.0400304982196));
#78675=CARTESIAN_POINT('Ctrl Pts',(19.6856656302613,-20.8513723491884,-21.0283736817803));
#78676=CARTESIAN_POINT('Ctrl Pts',(19.8417083679873,-20.7648076439597,-21.0188279067583));
#78677=CARTESIAN_POINT('Ctrl Pts',(20.0540512763229,-20.609244020643,-21.0045003305619));
#78678=CARTESIAN_POINT('Ctrl Pts',(20.1198668693067,-20.5546115656391,-20.9998169422385));
#78679=CARTESIAN_POINT('Ctrl Pts',(20.2094976760322,-20.4705508503281,-20.9927982572618));
#78680=CARTESIAN_POINT('Ctrl Pts',(20.2361143414899,-20.4442272596,-20.9906233506109));
#78681=CARTESIAN_POINT('Ctrl Pts',(20.2672420844694,-20.4117652877376,-20.9879473431042));
#78682=CARTESIAN_POINT('Ctrl Pts',(20.2724374979456,-20.4062888454141,-20.9874960908837));
#78683=CARTESIAN_POINT('Ctrl Pts',(20.2804620690263,-20.3977390903764,-20.9867916868579));
#78684=CARTESIAN_POINT('Ctrl Pts',(20.2833116672582,-20.3946849293539,-20.9865400749659));
#78685=CARTESIAN_POINT('Ctrl Pts',(20.2885756885573,-20.3890094395748,-20.986072495382));
#78686=CARTESIAN_POINT('Ctrl Pts',(20.2909925384615,-20.3863904403859,-20.9858567178472));
#78687=CARTESIAN_POINT('Ctrl Pts',(20.2964366074389,-20.3804610496373,-20.9853681829381));
#78688=CARTESIAN_POINT('Ctrl Pts',(20.2994599073349,-20.3771471503904,-20.9850951364374));
#78689=CARTESIAN_POINT('Ctrl Pts',(20.3083384151675,-20.3673529006457,-20.9842881916601));
#78690=CARTESIAN_POINT('Ctrl Pts',(20.3141639959375,-20.3608459882982,-20.9837521483915));
#78691=CARTESIAN_POINT('Ctrl Pts',(20.35555109441,-20.3140388342587,-20.9798977671729));
#78692=CARTESIAN_POINT('Ctrl Pts',(20.3896037507722,-20.272436632768,-20.9764808890683));
#78693=CARTESIAN_POINT('Ctrl Pts',(20.5153555542102,-20.1062850790474,-20.963010250249));
#78694=CARTESIAN_POINT('Ctrl Pts',(20.5948877805355,-19.9731278325685,-20.9526197441071));
#78695=CARTESIAN_POINT('Ctrl Pts',(20.6978946004503,-19.7479012118729,-20.9365438462385));
#78696=CARTESIAN_POINT('Ctrl Pts',(20.7309677614263,-19.6608472764353,-20.930640761115));
#78697=CARTESIAN_POINT('Ctrl Pts',(20.7643902521413,-19.5517081693673,-20.9236315561303));
#78698=CARTESIAN_POINT('Ctrl Pts',(20.7702684340306,-19.5314353972673,-20.9223453115321));
#78699=CARTESIAN_POINT('Ctrl Pts',(20.7782090523954,-19.5024349587697,-20.9205270526351));
#78700=CARTESIAN_POINT('Ctrl Pts',(20.7805206049522,-19.4937773630344,-20.9199869767051));
#78701=CARTESIAN_POINT('Ctrl Pts',(20.7844182241569,-19.4787984199277,-20.9190572054619));
#78702=CARTESIAN_POINT('Ctrl Pts',(20.786030185184,-19.4724839956821,-20.9186666759323));
#78703=CARTESIAN_POINT('Ctrl Pts',(20.7890639105027,-19.4603670061292,-20.9179199535675));
#78704=CARTESIAN_POINT('Ctrl Pts',(20.7904903183595,-19.4545656780874,-20.917563613984));
#78705=CARTESIAN_POINT('Ctrl Pts',(20.7941422189614,-19.439437159926,-20.9166373747414));
#78706=CARTESIAN_POINT('Ctrl Pts',(20.7963289478639,-19.4301006825188,-20.9160687273879));
#78707=CARTESIAN_POINT('Ctrl Pts',(20.8036013246229,-19.3980719070197,-20.9141279054184));
#78708=CARTESIAN_POINT('Ctrl Pts',(20.8083765840992,-19.3753103346977,-20.9127656733812));
#78709=CARTESIAN_POINT('Ctrl Pts',(20.8452419952168,-19.1839497769598,-20.9014445826094));
#78710=CARTESIAN_POINT('Ctrl Pts',(20.8570962745385,-19.0121042519913,-20.8921988008969));
#78711=CARTESIAN_POINT('Ctrl Pts',(20.8433537383876,-18.7510767321435,-20.8779847795815));
#78712=CARTESIAN_POINT('Ctrl Pts',(20.8329414366662,-18.6618523809092,-20.8730801985421));
#78713=CARTESIAN_POINT('Ctrl Pts',(20.8100173192434,-18.5356780504849,-20.8657635877288));
#78714=CARTESIAN_POINT('Ctrl Pts',(20.8021016158896,-18.497987707128,-20.8635279236192));
#78715=CARTESIAN_POINT('Ctrl Pts',(20.7913965946638,-18.4531351286419,-20.8607845954464));
#78716=CARTESIAN_POINT('Ctrl Pts',(20.7895901299587,-18.4457430284501,-20.8603297510928));
#78717=CARTESIAN_POINT('Ctrl Pts',(20.786727235976,-18.4342959800424,-20.8596209514185));
#78718=CARTESIAN_POINT('Ctrl Pts',(20.785698533698,-18.4302340719048,-20.8593685673205));
#78719=CARTESIAN_POINT('Ctrl Pts',(20.783772814819,-18.4227239828828,-20.8589002740831));
#78720=CARTESIAN_POINT('Ctrl Pts',(20.7828791498592,-18.4192750021244,-20.8586845597255));
#78721=CARTESIAN_POINT('Ctrl Pts',(20.7808448361325,-18.4115046792871,-20.8581971019553));
#78722=CARTESIAN_POINT('Ctrl Pts',(20.7796992137111,-18.4071847092005,-20.8579250751033));
#78723=CARTESIAN_POINT('Ctrl Pts',(20.7762947715889,-18.3945092076618,-20.8571239696015));
#78724=CARTESIAN_POINT('Ctrl Pts',(20.7739984095908,-18.3861639808309,-20.8565927917065));
#78725=CARTESIAN_POINT('Ctrl Pts',(20.7575867030867,-18.3279207456179,-20.8528604603406));
#78726=CARTESIAN_POINT('Ctrl Pts',(20.7416944489696,-18.2785461417397,-20.8495675614366));
#78727=CARTESIAN_POINT('Ctrl Pts',(20.7166531857815,-18.2095445505901,-20.8448281378035));
#78728=CARTESIAN_POINT('Ctrl Pts',(20.7089899557182,-18.1893936925551,-20.8434269961101));
#78729=CARTESIAN_POINT('Ctrl Pts',(20.6839298885056,-18.1264095481897,-20.839000316131));
#78730=CARTESIAN_POINT('Ctrl Pts',(20.6654372282101,-18.0840275359166,-20.8359523796574));
#78731=CARTESIAN_POINT('Ctrl Pts',(20.5985795379597,-17.9435401747494,-20.8256748341888));
#78732=CARTESIAN_POINT('Ctrl Pts',(20.5440021712157,-17.8485763827665,-20.8184438751073));
#78733=CARTESIAN_POINT('Ctrl Pts',(20.4512734533136,-17.7127688611721,-20.8078740102934));
#78734=CARTESIAN_POINT('Ctrl Pts',(20.4184542417522,-17.6685138660085,-20.8043867223197));
#78735=CARTESIAN_POINT('Ctrl Pts',(20.3624588554348,-17.5988604549313,-20.798831714606));
#78736=CARTESIAN_POINT('Ctrl Pts',(20.3403266229736,-17.5726596255167,-20.7967256035217));
#78737=CARTESIAN_POINT('Ctrl Pts',(20.3103939648875,-17.5389225539677,-20.7939898698394));
#78738=CARTESIAN_POINT('Ctrl Pts',(20.3031594613637,-17.5308932508023,-20.7933369250034));
#78739=CARTESIAN_POINT('Ctrl Pts',(20.2912071369385,-17.5178303740107,-20.7922714805455));
#78740=CARTESIAN_POINT('Ctrl Pts',(20.2865257041073,-17.5127639098186,-20.791857452064));
#78741=CARTESIAN_POINT('Ctrl Pts',(20.2774141969953,-17.5029992018415,-20.791057900251));
#78742=CARTESIAN_POINT('Ctrl Pts',(20.2729872313962,-17.4982981737729,-20.7906722507226));
#78743=CARTESIAN_POINT('Ctrl Pts',(20.2627134842322,-17.4874879351667,-20.7897837131695));
#78744=CARTESIAN_POINT('Ctrl Pts',(20.2568514447301,-17.4813933274447,-20.7892814915424));
#78745=CARTESIAN_POINT('Ctrl Pts',(20.2409826754627,-17.4650916208797,-20.7879345617977));
#78746=CARTESIAN_POINT('Ctrl Pts',(20.2309087182202,-17.4549503627865,-20.7870927968686));
#78747=CARTESIAN_POINT('Ctrl Pts',(20.1373585324325,-17.3626637221725,-20.7793944133068));
#78748=CARTESIAN_POINT('Ctrl Pts',(20.0472983860005,-17.2874707532506,-20.772856086988));
#78749=CARTESIAN_POINT('Ctrl Pts',(19.8174082193721,-17.1258649205835,-20.7574736519427));
#78750=CARTESIAN_POINT('Ctrl Pts',(19.6728755528101,-17.0475202675859,-20.7488161747321));
#78751=CARTESIAN_POINT('Ctrl Pts',(19.4917873481704,-16.9750269574099,-20.7376001066905));
#78752=CARTESIAN_POINT('Ctrl Pts',(19.4625462434253,-16.96406533958,-20.7357770075369));
#78753=CARTESIAN_POINT('Ctrl Pts',(19.4263259399395,-16.9513938616092,-20.7334917899725));
#78754=CARTESIAN_POINT('Ctrl Pts',(19.4195648475323,-16.9490669096079,-20.733064074883));
#78755=CARTESIAN_POINT('Ctrl Pts',(19.4089178832912,-16.9454627884744,-20.7323885498455));
#78756=CARTESIAN_POINT('Ctrl Pts',(19.4050398047849,-16.9441625289466,-20.7321420823351));
#78757=CARTESIAN_POINT('Ctrl Pts',(19.3977650651089,-16.9417468517903,-20.7316789284496));
#78758=CARTESIAN_POINT('Ctrl Pts',(19.3943693385109,-16.9406287966596,-20.7314624001223));
#78759=CARTESIAN_POINT('Ctrl Pts',(19.3865863945297,-16.9380880681282,-20.730965362684));
#78760=CARTESIAN_POINT('Ctrl Pts',(19.3821973626667,-16.9366711311145,-20.7306845213098));
#78761=CARTESIAN_POINT('Ctrl Pts',(19.3686045361586,-16.9323318755351,-20.729813141699));
#78762=CARTESIAN_POINT('Ctrl Pts',(19.3593855013232,-16.9294582286346,-20.7292198629124));
#78763=CARTESIAN_POINT('Ctrl Pts',(19.2481011210076,-16.8956035861596,-20.7220335718439));
#78764=CARTESIAN_POINT('Ctrl Pts',(19.143866171573,-16.8723196181018,-20.7150595624586));
#78765=CARTESIAN_POINT('Ctrl Pts',(18.9301039790352,-16.8412670820782,-20.7008100918327));
#78766=CARTESIAN_POINT('Ctrl Pts',(18.8208096022208,-16.8339544122939,-20.6935551844458));
#78767=CARTESIAN_POINT('Ctrl Pts',(18.6488221980256,-16.8357876682644,-20.6824362378933));
#78768=CARTESIAN_POINT('Ctrl Pts',(18.5862650049345,-16.8392327544126,-20.6784512271599));
#78769=CARTESIAN_POINT('Ctrl Pts',(18.4991746732176,-16.8479168578278,-20.6729961131759));
#78770=CARTESIAN_POINT('Ctrl Pts',(18.4744464032588,-16.8508239445997,-20.6714575295445));
#78771=CARTESIAN_POINT('Ctrl Pts',(18.4312406014699,-16.8566776976592,-20.6687868410496));
#78772=CARTESIAN_POINT('Ctrl Pts',(18.4127405261699,-16.8594343045438,-20.6676489548771));
#78773=CARTESIAN_POINT('Ctrl Pts',(18.3858544828323,-16.8638054338338,-20.6660030997113));
#78774=CARTESIAN_POINT('Ctrl Pts',(18.3774382982314,-16.8652260296202,-20.665489014493));
#78775=CARTESIAN_POINT('Ctrl Pts',(18.3626811148188,-16.8678088284576,-20.6645895033053));
#78776=CARTESIAN_POINT('Ctrl Pts',(18.356336447432,-16.8689491613225,-20.6642033878881));
#78777=CARTESIAN_POINT('Ctrl Pts',(18.3440146591901,-16.8712219146808,-20.6634546912562));
#78778=CARTESIAN_POINT('Ctrl Pts',(18.3380370223699,-16.8723511527362,-20.6630920129195));
#78779=CARTESIAN_POINT('Ctrl Pts',(18.3237394707411,-16.8751159896875,-20.6622257846882));
#78780=CARTESIAN_POINT('Ctrl Pts',(18.3154243103936,-16.8767758459848,-20.6617230119399));
#78781=CARTESIAN_POINT('Ctrl Pts',(18.2853398289162,-16.8829694302244,-20.6599074343806));
#78782=CARTESIAN_POINT('Ctrl Pts',(18.2636318237767,-16.8877962111729,-20.6586039828981));
#78783=CARTESIAN_POINT('Ctrl Pts',(18.0627480347725,-16.9357964304618,-20.6465932324424));
#78784=CARTESIAN_POINT('Ctrl Pts',(17.8898576569068,-17.0018497835049,-20.6367285525924));
#78785=CARTESIAN_POINT('Ctrl Pts',(17.6564347876173,-17.1279653232637,-20.6222691800986));
#78786=CARTESIAN_POINT('Ctrl Pts',(17.5874485019967,-17.1705211486931,-20.6178175296491));
#78787=CARTESIAN_POINT('Ctrl Pts',(17.4913574344798,-17.2376945439702,-20.6111127763509));
#78788=CARTESIAN_POINT('Ctrl Pts',(17.4621800954307,-17.2592278600716,-20.6090040722916));
#78789=CARTESIAN_POINT('Ctrl Pts',(17.4276696901645,-17.2860930182023,-20.6064014668105));
#78790=CARTESIAN_POINT('Ctrl Pts',(17.4217917968494,-17.2907189948134,-20.6059542803094));
#78791=CARTESIAN_POINT('Ctrl Pts',(17.412681517766,-17.2979674147469,-20.6052548570601));
#78792=CARTESIAN_POINT('Ctrl Pts',(17.4094320752328,-17.300568458408,-20.6050041252277));
#78793=CARTESIAN_POINT('Ctrl Pts',(17.4034133424525,-17.3054153954806,-20.6045373169608));
#78794=CARTESIAN_POINT('Ctrl Pts',(17.4006420477552,-17.3076587082765,-20.6043214252069));
#78795=CARTESIAN_POINT('Ctrl Pts',(17.3943809871138,-17.3127531584176,-20.6038315160248));
#78796=CARTESIAN_POINT('Ctrl Pts',(17.3908946677011,-17.3156084292549,-20.6035572024839));
#78797=CARTESIAN_POINT('Ctrl Pts',(17.3806055013101,-17.3240902151048,-20.6027431824962));
#78798=CARTESIAN_POINT('Ctrl Pts',(17.3738288014987,-17.3297480955845,-20.6022012760981));
#78799=CARTESIAN_POINT('Ctrl Pts',(17.3242100279993,-17.3717043760233,-20.5981920227039));
#78800=CARTESIAN_POINT('Ctrl Pts',(17.2827955738554,-17.4096490180562,-20.5946171851587));
#78801=CARTESIAN_POINT('Ctrl Pts',(17.1985927881025,-17.4931933656554,-20.5869375005044));
#78802=CARTESIAN_POINT('Ctrl Pts',(17.1562146413819,-17.5391359405585,-20.5828222616848));
#78803=CARTESIAN_POINT('Ctrl Pts',(17.0452480438396,-17.670664243137,-20.5714553749442));
#78804=CARTESIAN_POINT('Ctrl Pts',(16.9811726594501,-17.7598153394788,-20.5642057657625));
#78805=CARTESIAN_POINT('Ctrl Pts',(16.8955510661131,-17.9008760083811,-20.5535967706378));
#78806=CARTESIAN_POINT('Ctrl Pts',(16.868681749659,-17.9493311682977,-20.5500891263359));
#78807=CARTESIAN_POINT('Ctrl Pts',(16.8282391527538,-18.0295304688711,-20.5445055504034));
#78808=CARTESIAN_POINT('Ctrl Pts',(16.8134880190854,-18.0606479973414,-20.5423907290272));
#78809=CARTESIAN_POINT('Ctrl Pts',(16.7951057144783,-18.1020028912704,-20.5396455447155));
#78810=CARTESIAN_POINT('Ctrl Pts',(16.7907854902543,-18.1119264846431,-20.5389916547816));
#78811=CARTESIAN_POINT('Ctrl Pts',(16.7838354324334,-18.1282313523914,-20.5379250851755));
#78812=CARTESIAN_POINT('Ctrl Pts',(16.7811604048282,-18.134593037307,-20.5375108700528));
#78813=CARTESIAN_POINT('Ctrl Pts',(16.7760434384849,-18.1469305777582,-20.5367112457338));
#78814=CARTESIAN_POINT('Ctrl Pts',(16.773597634443,-18.152904737874,-20.5363257088402));
#78815=CARTESIAN_POINT('Ctrl Pts',(16.768014752243,-18.1667214821484,-20.5354378421266));
#78816=CARTESIAN_POINT('Ctrl Pts',(16.7648971947904,-18.1745718742755,-20.5349361757676));
#78817=CARTESIAN_POINT('Ctrl Pts',(16.7566421279101,-18.1957273913413,-20.5335916482684));
#78818=CARTESIAN_POINT('Ctrl Pts',(16.7515918944921,-18.2090662674463,-20.5327517142581));
#78819=CARTESIAN_POINT('Ctrl Pts',(16.6965077126158,-18.3591188847362,-20.5233871995423));
#78820=CARTESIAN_POINT('Ctrl Pts',(16.6605663579691,-18.5005981038488,-20.5153746929697));
#78821=CARTESIAN_POINT('Ctrl Pts',(16.6244283768297,-18.7468873155227,-20.5018389966347));
#78822=CARTESIAN_POINT('Ctrl Pts',(16.6169334233456,-18.8500661998662,-20.4962757985682));
#78823=CARTESIAN_POINT('Ctrl Pts',(16.6170394068497,-19.0134280313683,-20.4871374011508));
#78824=CARTESIAN_POINT('Ctrl Pts',(16.6196337803259,-19.0734481173039,-20.4837076718875));
#78825=CARTESIAN_POINT('Ctrl Pts',(16.6255428349298,-19.1422045998558,-20.4796144300126));
#78826=CARTESIAN_POINT('Ctrl Pts',(16.6263673828061,-19.1511335011068,-20.4790796667383));
#78827=CARTESIAN_POINT('Ctrl Pts',(16.6276944058085,-19.1645707388497,-20.478269705438));
#78828=CARTESIAN_POINT('Ctrl Pts',(16.6281546998097,-19.1690832695645,-20.4779968197555));
#78829=CARTESIAN_POINT('Ctrl Pts',(16.6290029491409,-19.1771425004653,-20.4775078228937));
#78830=CARTESIAN_POINT('Ctrl Pts',(16.629385371026,-19.1806897306192,-20.4772920256087));
#78831=CARTESIAN_POINT('Ctrl Pts',(16.6302310228456,-19.1883519364266,-20.4768246509355));
#78832=CARTESIAN_POINT('Ctrl Pts',(16.6306973530491,-19.192466466978,-20.4765729065439));
#78833=CARTESIAN_POINT('Ctrl Pts',(16.6320285817753,-19.2039119860905,-20.475870531854));
#78834=CARTESIAN_POINT('Ctrl Pts',(16.6329197476738,-19.2112397758109,-20.4754184619776));
#78835=CARTESIAN_POINT('Ctrl Pts',(16.6382144752587,-19.2529550243667,-20.4728319164278));
#78836=CARTESIAN_POINT('Ctrl Pts',(16.643423628833,-19.2872327656516,-20.4706561137669));
#78837=CARTESIAN_POINT('Ctrl Pts',(16.6625927921858,-19.3954148933767,-20.4636610241718));
#78838=CARTESIAN_POINT('Ctrl Pts',(16.6796496226979,-19.4687083943756,-20.45873241018));
#78839=CARTESIAN_POINT('Ctrl Pts',(16.7139659294228,-19.5871935575331,-20.4505956064325));
#78840=CARTESIAN_POINT('Ctrl Pts',(16.7289275848391,-19.6329445735838,-20.4474103338749));
#78841=CARTESIAN_POINT('Ctrl Pts',(16.7454193204093,-19.6781101023665,-20.4442392291799));
#78842=CARTESIAN_POINT('Origin',(18.734,-18.952,0.));
#78843=CARTESIAN_POINT('',(16.7454194498907,-19.678110456974,-19.6425235871583));
#78844=CARTESIAN_POINT('',(16.7452305273115,-19.6781794125984,-19.8664843216556));
#78845=CARTESIAN_POINT('',(16.7454194499637,-19.6781104571739,0.));
#78846=CARTESIAN_POINT('',(16.6200797572234,-18.9511717419853,-19.9109991808971));
#78847=CARTESIAN_POINT('Ctrl Pts',(16.7452305273115,-19.6781794125984,-19.8664843216556));
#78848=CARTESIAN_POINT('Ctrl Pts',(16.6631151187494,-19.4459846869538,-19.8813041214296));
#78849=CARTESIAN_POINT('Ctrl Pts',(16.6210474187959,-19.1984405238965,-19.8961239212035));
#78850=CARTESIAN_POINT('Ctrl Pts',(16.6201759917111,-18.9511685861839,-19.9109437209775));
#78851=CARTESIAN_POINT('Ctrl Pts',(16.6170001249218,-18.9512727318511,-19.9127739724915));
#78852=CARTESIAN_POINT('Ctrl Pts',(16.6170670032748,-18.7565969919401,-19.9239833310404));
#78853=CARTESIAN_POINT('Ctrl Pts',(16.6439835682874,-18.5628628690705,-19.9342646472684));
#78854=CARTESIAN_POINT('Ctrl Pts',(16.7140733703376,-18.3151987866819,-19.9484105632264));
#78855=CARTESIAN_POINT('Ctrl Pts',(16.7338151550543,-18.2556675991902,-19.951902303785));
#78856=CARTESIAN_POINT('Ctrl Pts',(16.7671936907326,-18.1682155204606,-19.9572865138648));
#78857=CARTESIAN_POINT('Ctrl Pts',(16.7788510580608,-18.139573045479,-19.9590922814678));
#78858=CARTESIAN_POINT('Ctrl Pts',(16.793961811212,-18.1046561292592,-19.9613581669638));
#78859=CARTESIAN_POINT('Ctrl Pts',(16.7968258157541,-18.0981288236282,-19.9617845621696));
#78860=CARTESIAN_POINT('Ctrl Pts',(16.8013829440265,-18.0878836865476,-19.962458450798));
#78861=CARTESIAN_POINT('Ctrl Pts',(16.8030539889759,-18.0841560105205,-19.9627046122851));
#78862=CARTESIAN_POINT('Ctrl Pts',(16.8062079245958,-18.0771745888939,-19.9631674992383));
#78863=CARTESIAN_POINT('Ctrl Pts',(16.8076882729554,-18.0739197556721,-19.963384068519));
#78864=CARTESIAN_POINT('Ctrl Pts',(16.8111000205154,-18.0664685160747,-19.9638816023128));
#78865=CARTESIAN_POINT('Ctrl Pts',(16.8130369085069,-18.062274682662,-19.9641629017101));
#78866=CARTESIAN_POINT('Ctrl Pts',(16.8190812886983,-18.0492988732612,-19.9650371083213));
#78867=CARTESIAN_POINT('Ctrl Pts',(16.8232353258609,-18.0405388944304,-19.9656327814039));
#78868=CARTESIAN_POINT('Ctrl Pts',(16.8705046782861,-17.9426012766077,-19.9723517442861));
#78869=CARTESIAN_POINT('Ctrl Pts',(16.9197630785505,-17.8565364755763,-19.9788044444127));
#78870=CARTESIAN_POINT('Ctrl Pts',(17.0685517912955,-17.6342992449471,-19.9964225358484));
#78871=CARTESIAN_POINT('Ctrl Pts',(17.1786301555595,-17.5060074329291,-20.007610743824));
#78872=CARTESIAN_POINT('Ctrl Pts',(17.3256262175747,-17.3711346946008,-20.0201376411174));
#78873=CARTESIAN_POINT('Ctrl Pts',(17.3489492164882,-17.350661088638,-20.0220662574656));
#78874=CARTESIAN_POINT('Ctrl Pts',(17.3843093416891,-17.3209716955516,-20.0249047609683));
#78875=CARTESIAN_POINT('Ctrl Pts',(17.3960081347465,-17.3113611030345,-20.025830467425));
#78876=CARTESIAN_POINT('Ctrl Pts',(17.414908947366,-17.2961706735294,-20.0273049894154));
#78877=CARTESIAN_POINT('Ctrl Pts',(17.4220454704626,-17.2905105236463,-20.027857017166));
#78878=CARTESIAN_POINT('Ctrl Pts',(17.4357263538302,-17.2798029908296,-20.0289063875791));
#78879=CARTESIAN_POINT('Ctrl Pts',(17.4422641581444,-17.2747475396626,-20.029404046488));
#78880=CARTESIAN_POINT('Ctrl Pts',(17.4537916361757,-17.2659411317145,-20.0302749183255));
#78881=CARTESIAN_POINT('Ctrl Pts',(17.4587685760821,-17.2621737429912,-20.0306487777281));
#78882=CARTESIAN_POINT('Ctrl Pts',(17.4686241248444,-17.2547817372316,-20.0313849420241));
#78883=CARTESIAN_POINT('Ctrl Pts',(17.473501821549,-17.2511560094449,-20.0317472882647));
#78884=CARTESIAN_POINT('Ctrl Pts',(17.4852043815327,-17.2425351623169,-20.0326119127962));
#78885=CARTESIAN_POINT('Ctrl Pts',(17.492043730996,-17.2375598123545,-20.0331134205157));
#78886=CARTESIAN_POINT('Ctrl Pts',(17.5168596014723,-17.2197336990024,-20.034919581753));
#78887=CARTESIAN_POINT('Ctrl Pts',(17.5350076330159,-17.2071233151211,-20.0362150101887));
#78888=CARTESIAN_POINT('Ctrl Pts',(17.7074294876819,-17.0912744087843,-20.0482965234404));
#78889=CARTESIAN_POINT('Ctrl Pts',(17.8744496948748,-17.0084655834537,-20.0582255373285));
#78890=CARTESIAN_POINT('Ctrl Pts',(18.1259660093946,-16.9226151349315,-20.072713585799));
#78891=CARTESIAN_POINT('Ctrl Pts',(18.2031933790864,-16.9010610467242,-20.0771197353448));
#78892=CARTESIAN_POINT('Ctrl Pts',(18.3166409704104,-16.876235516632,-20.0837626423482));
#78893=CARTESIAN_POINT('Ctrl Pts',(18.3520210311286,-16.8694346423479,-20.0858580509248));
#78894=CARTESIAN_POINT('Ctrl Pts',(18.3949201538196,-16.8623183023126,-20.0884459112971));
#78895=CARTESIAN_POINT('Ctrl Pts',(18.4022916952279,-16.8611355049851,-20.0888922652693));
#78896=CARTESIAN_POINT('Ctrl Pts',(18.4137793677927,-16.8593545340618,-20.0895906696082));
#78897=CARTESIAN_POINT('Ctrl Pts',(18.4178913501114,-16.8587294441031,-20.0898412222025));
#78898=CARTESIAN_POINT('Ctrl Pts',(18.4255321164967,-16.8575909471096,-20.0903078769221));
#78899=CARTESIAN_POINT('Ctrl Pts',(18.4290603652509,-16.857074336752,-20.0905237954991));
#78900=CARTESIAN_POINT('Ctrl Pts',(18.4370546676644,-16.8559244249816,-20.091013998559));
#78901=CARTESIAN_POINT('Ctrl Pts',(18.4415214277539,-16.8552964848385,-20.0912885806234));
#78902=CARTESIAN_POINT('Ctrl Pts',(18.4530601951649,-16.8537119466705,-20.0919996018318));
#78903=CARTESIAN_POINT('Ctrl Pts',(18.4601350276012,-16.8527768336195,-20.0924372080098));
#78904=CARTESIAN_POINT('Ctrl Pts',(18.5036224153015,-16.8472524836331,-20.0951366607305));
#78905=CARTESIAN_POINT('Ctrl Pts',(18.5401421550111,-16.843575303544,-20.0974447813846));
#78906=CARTESIAN_POINT('Ctrl Pts',(18.7466342443177,-16.828193311188,-20.1106595079955));
#78907=CARTESIAN_POINT('Ctrl Pts',(18.9174369828871,-16.8360915855324,-20.122154853729));
#78908=CARTESIAN_POINT('Ctrl Pts',(19.1796012984132,-16.8802268205788,-20.1394324934186));
#78909=CARTESIAN_POINT('Ctrl Pts',(19.2725816120223,-16.9024296220449,-20.1454987964668));
#78910=CARTESIAN_POINT('Ctrl Pts',(19.3841900256898,-16.9372047258563,-20.1526795589692));
#78911=CARTESIAN_POINT('Ctrl Pts',(19.404526438532,-16.9438811254705,-20.1539841317236));
#78912=CARTESIAN_POINT('Ctrl Pts',(19.4332771835243,-16.9538054070952,-20.1558235785827));
#78913=CARTESIAN_POINT('Ctrl Pts',(19.4417768933293,-16.9568002396486,-20.1563667706154));
#78914=CARTESIAN_POINT('Ctrl Pts',(19.4563991489929,-16.9620575214803,-20.1573002552613));
#78915=CARTESIAN_POINT('Ctrl Pts',(19.462530780882,-16.964294161333,-20.1576913994153));
#78916=CARTESIAN_POINT('Ctrl Pts',(19.4742457579964,-16.9686289324353,-20.1584381748218));
#78917=CARTESIAN_POINT('Ctrl Pts',(19.4798307625224,-16.9707223696108,-20.1587939582294));
#78918=CARTESIAN_POINT('Ctrl Pts',(19.4943187914687,-16.9762228857185,-20.1597163248234));
#78919=CARTESIAN_POINT('Ctrl Pts',(19.5032078468509,-16.9796665690507,-20.1602816771984));
#78920=CARTESIAN_POINT('Ctrl Pts',(19.5333783743245,-16.991589837711,-20.1621988857278));
#78921=CARTESIAN_POINT('Ctrl Pts',(19.554545808818,-17.000354943732,-20.1635411310891));
#78922=CARTESIAN_POINT('Ctrl Pts',(19.7375892096665,-17.0796550024494,-20.1751337316173));
#78923=CARTESIAN_POINT('Ctrl Pts',(19.8901913225283,-17.1698396917425,-20.1846222462391));
#78924=CARTESIAN_POINT('Ctrl Pts',(20.0980331049384,-17.3307226306215,-20.1989258069311));
#78925=CARTESIAN_POINT('Ctrl Pts',(20.1629359992613,-17.3876259465707,-20.2036494651612));
#78926=CARTESIAN_POINT('Ctrl Pts',(20.2509103524937,-17.4748107899274,-20.210722456218));
#78927=CARTESIAN_POINT('Ctrl Pts',(20.2769252789562,-17.5020047690118,-20.2129085690859));
#78928=CARTESIAN_POINT('Ctrl Pts',(20.3072788812218,-17.5354761826385,-20.2155970151179));
#78929=CARTESIAN_POINT('Ctrl Pts',(20.3123277196757,-17.5411039128815,-20.216048963388));
#78930=CARTESIAN_POINT('Ctrl Pts',(20.3201207742068,-17.5498846834153,-20.2167542318291));
#78931=CARTESIAN_POINT('Ctrl Pts',(20.3228860386396,-17.5530190755787,-20.2170060062323));
#78932=CARTESIAN_POINT('Ctrl Pts',(20.3279918658094,-17.558841131249,-20.2174737549519));
#78933=CARTESIAN_POINT('Ctrl Pts',(20.3303349310455,-17.5615265233791,-20.2176895382437));
#78934=CARTESIAN_POINT('Ctrl Pts',(20.3356101175626,-17.5676033334991,-20.2181779155151));
#78935=CARTESIAN_POINT('Ctrl Pts',(20.3385382365935,-17.5709981370934,-20.2184507976054));
#78936=CARTESIAN_POINT('Ctrl Pts',(20.347130010663,-17.5810234829829,-20.2192567391577));
#78937=CARTESIAN_POINT('Ctrl Pts',(20.3527634259066,-17.5876796540211,-20.2197919354018));
#78938=CARTESIAN_POINT('Ctrl Pts',(20.3925711869254,-17.6353082184688,-20.223621106529));
#78939=CARTESIAN_POINT('Ctrl Pts',(20.4252240993812,-17.6775214247544,-20.2270121780518));
#78940=CARTESIAN_POINT('Ctrl Pts',(20.4665317681763,-17.7353095726767,-20.2316030525249));
#78941=CARTESIAN_POINT('Ctrl Pts',(20.476637704108,-17.7498287429233,-20.2327524135595));
#78942=CARTESIAN_POINT('Ctrl Pts',(20.5137223988464,-17.804558563249,-20.2370653467181));
#78943=CARTESIAN_POINT('Ctrl Pts',(20.5395005206388,-17.8455636931513,-20.240257472366));
#78944=CARTESIAN_POINT('Ctrl Pts',(20.6188548644469,-17.9819610211768,-20.2506814207805));
#78945=CARTESIAN_POINT('Ctrl Pts',(20.6664543604433,-18.0806349266119,-20.257914189928));
#78946=CARTESIAN_POINT('Ctrl Pts',(20.7262435630295,-18.2338839091239,-20.2684877851117));
#78947=CARTESIAN_POINT('Ctrl Pts',(20.7442601962116,-18.2859820580437,-20.2719769904407));
#78948=CARTESIAN_POINT('Ctrl Pts',(20.7701619245909,-18.3715602124066,-20.2775346482309));
#78949=CARTESIAN_POINT('Ctrl Pts',(20.7793002214434,-18.404630882613,-20.2796415418738));
#78950=CARTESIAN_POINT('Ctrl Pts',(20.7902558916234,-18.448395463685,-20.2823780938825));
#78951=CARTESIAN_POINT('Ctrl Pts',(20.7928002840516,-18.4589003974776,-20.2830310946352));
#78952=CARTESIAN_POINT('Ctrl Pts',(20.7968365494926,-18.476140828162,-20.2840965852931));
#78953=CARTESIAN_POINT('Ctrl Pts',(20.7983761272019,-18.4828648504576,-20.2845106046632));
#78954=CARTESIAN_POINT('Ctrl Pts',(20.8012931086656,-18.4958970611322,-20.2853101075458));
#78955=CARTESIAN_POINT('Ctrl Pts',(20.8026745699498,-18.5022042540793,-20.2856957174105));
#78956=CARTESIAN_POINT('Ctrl Pts',(20.8057982531238,-18.5167845639653,-20.2865841184869));
#78957=CARTESIAN_POINT('Ctrl Pts',(20.8075198215551,-18.5250620300429,-20.287086243667));
#78958=CARTESIAN_POINT('Ctrl Pts',(20.812017578788,-18.547356791025,-20.2884328133981));
#78959=CARTESIAN_POINT('Ctrl Pts',(20.8147015409593,-18.5613924006362,-20.2892743167176));
#78960=CARTESIAN_POINT('Ctrl Pts',(20.8380201065115,-18.690402646008,-20.2969546320946));
#78961=CARTESIAN_POINT('Ctrl Pts',(20.8492492306908,-18.8068802661364,-20.3034769044381));
#78962=CARTESIAN_POINT('Ctrl Pts',(20.8529854711163,-19.086379167592,-20.3187794026293));
#78963=CARTESIAN_POINT('Ctrl Pts',(20.8364007118598,-19.2487433283176,-20.3273767148595));
#78964=CARTESIAN_POINT('Ctrl Pts',(20.7943880542967,-19.4393918140765,-20.3385853422936));
#78965=CARTESIAN_POINT('Ctrl Pts',(20.7866465694543,-19.4710293951073,-20.3404848059556));
#78966=CARTESIAN_POINT('Ctrl Pts',(20.776295418608,-19.5094682892352,-20.3428550035646));
#78967=CARTESIAN_POINT('Ctrl Pts',(20.7743760315172,-19.5164529359754,-20.3432882285365));
#78968=CARTESIAN_POINT('Ctrl Pts',(20.7713113379336,-19.5273854437378,-20.3439705081739));
#78969=CARTESIAN_POINT('Ctrl Pts',(20.7701902932699,-19.5313401293462,-20.3442181750627));
#78970=CARTESIAN_POINT('Ctrl Pts',(20.7680736334476,-19.5387249876467,-20.3446823151683));
#78971=CARTESIAN_POINT('Ctrl Pts',(20.7670808527248,-19.5421559141823,-20.3448986226805));
#78972=CARTESIAN_POINT('Ctrl Pts',(20.7647951982406,-19.5499806348931,-20.3453934712168));
#78973=CARTESIAN_POINT('Ctrl Pts',(20.7634967497832,-19.5543727405959,-20.3456723336393));
#78974=CARTESIAN_POINT('Ctrl Pts',(20.7594632334565,-19.5678553468216,-20.3465316703975));
#78975=CARTESIAN_POINT('Ctrl Pts',(20.7566813079152,-19.5769315460023,-20.3471147793858));
#78976=CARTESIAN_POINT('Ctrl Pts',(20.731215296637,-19.6580642910096,-20.3523667852692));
#78977=CARTESIAN_POINT('Ctrl Pts',(20.7047527302255,-19.7288699272416,-20.3572289299204));
#78978=CARTESIAN_POINT('Ctrl Pts',(20.6204510971423,-19.9222190009485,-20.3710221902335));
#78979=CARTESIAN_POINT('Ctrl Pts',(20.5545471961497,-20.0408683284741,-20.3800726728836));
#78980=CARTESIAN_POINT('Ctrl Pts',(20.4267722956368,-20.2264792167476,-20.3946760285343));
#78981=CARTESIAN_POINT('Ctrl Pts',(20.3711100367118,-20.2972321902289,-20.4003745739396));
#78982=CARTESIAN_POINT('Ctrl Pts',(20.2972801652681,-20.3796812855696,-20.4071681931084));
#78983=CARTESIAN_POINT('Ctrl Pts',(20.2832249262702,-20.3949209625224,-20.4084311939097));
#78984=CARTESIAN_POINT('Ctrl Pts',(20.2628205713741,-20.4164028865192,-20.4102226329144));
#78985=CARTESIAN_POINT('Ctrl Pts',(20.2566527608454,-20.4228149874029,-20.4107588101116));
#78986=CARTESIAN_POINT('Ctrl Pts',(20.2459048569644,-20.4338485187958,-20.411684034936));
#78987=CARTESIAN_POINT('Ctrl Pts',(20.2413435782436,-20.4384880314903,-20.4120738945192));
#78988=CARTESIAN_POINT('Ctrl Pts',(20.232542542238,-20.447357856229,-20.4128208272488));
#78989=CARTESIAN_POINT('Ctrl Pts',(20.2283060856346,-20.4515913418839,-20.413178040014));
#78990=CARTESIAN_POINT('Ctrl Pts',(20.2171839624836,-20.4626117323176,-20.4141098208219));
#78991=CARTESIAN_POINT('Ctrl Pts',(20.2102696182567,-20.4693695961458,-20.4146831069051));
#78992=CARTESIAN_POINT('Ctrl Pts',(20.1862282668145,-20.4925469743607,-20.41665618853));
#78993=CARTESIAN_POINT('Ctrl Pts',(20.1688713023723,-20.5087261581908,-20.4180455865978));
#78994=CARTESIAN_POINT('Ctrl Pts',(20.0307849583594,-20.6331703426115,-20.4288393372118));
#78995=CARTESIAN_POINT('Ctrl Pts',(19.8982501185042,-20.7275319192425,-20.4376181142168));
#78996=CARTESIAN_POINT('Ctrl Pts',(19.6420170131075,-20.8688214622892,-20.4535141852791));
#78997=CARTESIAN_POINT('Ctrl Pts',(19.5222459529865,-20.9211007722441,-20.4606069961755));
#78998=CARTESIAN_POINT('Ctrl Pts',(19.3871569990757,-20.9657567789928,-20.4690032984038));
#78999=CARTESIAN_POINT('Ctrl Pts',(19.3758345350771,-20.9693940728918,-20.4697100401756));
#79000=CARTESIAN_POINT('Ctrl Pts',(19.3596901468902,-20.9744307256799,-20.4707228226114));
#79001=CARTESIAN_POINT('Ctrl Pts',(19.354892725446,-20.9759086991256,-20.4710244104664));
#79002=CARTESIAN_POINT('Ctrl Pts',(19.3466142517837,-20.9784268993233,-20.4715459942964));
#79003=CARTESIAN_POINT('Ctrl Pts',(19.3431356587079,-20.9794752646904,-20.4717655155993));
#79004=CARTESIAN_POINT('Ctrl Pts',(19.3363840691346,-20.9814910893136,-20.4721922948394));
#79005=CARTESIAN_POINT('Ctrl Pts',(19.3331114250735,-20.9824595904165,-20.4723994845306));
#79006=CARTESIAN_POINT('Ctrl Pts',(19.3242721818198,-20.9850522316033,-20.4729599300098));
#79007=CARTESIAN_POINT('Ctrl Pts',(19.3187012761245,-20.9866614069513,-20.4733140433683));
#79008=CARTESIAN_POINT('Ctrl Pts',(19.2979807360501,-20.9925544819296,-20.4746342746687));
#79009=CARTESIAN_POINT('Ctrl Pts',(19.2827905008595,-20.996692108103,-20.4756083480782));
#79010=CARTESIAN_POINT('Ctrl Pts',(19.140118424596,-21.0338498396404,-20.4848060651902));
#79011=CARTESIAN_POINT('Ctrl Pts',(19.0098734654943,-21.0550736190206,-20.4935482954804));
#79012=CARTESIAN_POINT('Ctrl Pts',(18.7196143114129,-21.0749342222452,-20.512766475312));
#79013=CARTESIAN_POINT('Ctrl Pts',(18.5599657294328,-21.0678418905443,-20.523135291233));
#79014=CARTESIAN_POINT('Ctrl Pts',(18.3815824983642,-21.0395688654763,-20.534228098973));
#79015=CARTESIAN_POINT('Ctrl Pts',(18.360615121053,-21.0359207392878,-20.5355251355653));
#79016=CARTESIAN_POINT('Ctrl Pts',(18.330871681186,-21.0302823202987,-20.5373559108369));
#79017=CARTESIAN_POINT('Ctrl Pts',(18.3220483193726,-21.0285513865597,-20.5378978604425));
#79018=CARTESIAN_POINT('Ctrl Pts',(18.3068429916011,-21.0254677339177,-20.5388298955764));
#79019=CARTESIAN_POINT('Ctrl Pts',(18.3004558100196,-21.0241416433813,-20.5392208254853));
#79020=CARTESIAN_POINT('Ctrl Pts',(18.2882360762416,-21.0215456394119,-20.5399676584656));
#79021=CARTESIAN_POINT('Ctrl Pts',(18.282402575381,-21.0202805410617,-20.5403237114558));
#79022=CARTESIAN_POINT('Ctrl Pts',(18.2672432337545,-21.0169257752085,-20.5412477862828));
#79023=CARTESIAN_POINT('Ctrl Pts',(18.2579259873522,-21.01479758459,-20.541814568264));
#79024=CARTESIAN_POINT('Ctrl Pts',(18.2261825279712,-21.0073204000864,-20.5437418099668));
#79025=CARTESIAN_POINT('Ctrl Pts',(18.2038289350488,-21.0016680792794,-20.5450925203369));
#79026=CARTESIAN_POINT('Ctrl Pts',(18.013003279222,-20.9500851485518,-20.556578377997));
#79027=CARTESIAN_POINT('Ctrl Pts',(17.850721595277,-20.8838401927936,-20.5659712706361));
#79028=CARTESIAN_POINT('Ctrl Pts',(17.6219933391388,-20.7555536562888,-20.5802385231723));
#79029=CARTESIAN_POINT('Ctrl Pts',(17.5483208739786,-20.7079974898499,-20.5850329556423));
#79030=CARTESIAN_POINT('Ctrl Pts',(17.4472442349054,-20.6334847078711,-20.5922013750864));
#79031=CARTESIAN_POINT('Ctrl Pts',(17.4172900622693,-20.6101332147852,-20.594407074953));
#79032=CARTESIAN_POINT('Ctrl Pts',(17.3821312054603,-20.5811707177156,-20.59711723556));
#79033=CARTESIAN_POINT('Ctrl Pts',(17.3763062266334,-20.5763195741404,-20.5975703609094));
#79034=CARTESIAN_POINT('Ctrl Pts',(17.367306706735,-20.5687423883025,-20.5982770759198));
#79035=CARTESIAN_POINT('Ctrl Pts',(17.3641139141255,-20.5660379856191,-20.5985291096791));
#79036=CARTESIAN_POINT('Ctrl Pts',(17.3582169705406,-20.5610129749576,-20.5989970811449));
#79037=CARTESIAN_POINT('Ctrl Pts',(17.3555106532072,-20.5586949984157,-20.5992128261797));
#79038=CARTESIAN_POINT('Ctrl Pts',(17.3494172470552,-20.5534492325401,-20.5997007904362));
#79039=CARTESIAN_POINT('Ctrl Pts',(17.3460336063529,-20.5505175424153,-20.5999732956908));
#79040=CARTESIAN_POINT('Ctrl Pts',(17.3361072837873,-20.5418617945954,-20.6007772011956));
#79041=CARTESIAN_POINT('Ctrl Pts',(17.3295906231659,-20.5361082249202,-20.6013107229349));
#79042=CARTESIAN_POINT('Ctrl Pts',(17.2837289770084,-20.4951114914313,-20.6051052078611));
#79043=CARTESIAN_POINT('Ctrl Pts',(17.2456829977284,-20.4584496693645,-20.6084613702442));
#79044=CARTESIAN_POINT('Ctrl Pts',(17.1955082977119,-20.406342978521,-20.6131348438562));
#79045=CARTESIAN_POINT('Ctrl Pts',(17.1821608933518,-20.3920922093448,-20.6144037584559));
#79046=CARTESIAN_POINT('Ctrl Pts',(17.0704030636719,-20.2694124175078,-20.6252363405281));
#79047=CARTESIAN_POINT('Ctrl Pts',(16.98328057628,-20.1512151403582,-20.6350415616551));
#79048=CARTESIAN_POINT('Ctrl Pts',(16.8777709685967,-19.9717612418561,-20.6484905953123));
#79049=CARTESIAN_POINT('Ctrl Pts',(16.8488257015203,-19.9172037082465,-20.6524167066091));
#79050=CARTESIAN_POINT('Ctrl Pts',(16.8063135223856,-19.8278420853232,-20.658582707094));
#79051=CARTESIAN_POINT('Ctrl Pts',(16.7912114312221,-19.7938119548773,-20.6608723687523));
#79052=CARTESIAN_POINT('Ctrl Pts',(16.7727688488821,-19.7491105654178,-20.6638069414725));
#79053=CARTESIAN_POINT('Ctrl Pts',(16.7686050596556,-19.7387881655802,-20.6644796308978));
#79054=CARTESIAN_POINT('Ctrl Pts',(16.7619670948561,-19.7219505040658,-20.6655689931111));
#79055=CARTESIAN_POINT('Ctrl Pts',(16.759443381107,-19.7154551187033,-20.6659873301411));
#79056=CARTESIAN_POINT('Ctrl Pts',(16.754652614013,-19.7029422564804,-20.6667896188495));
#79057=CARTESIAN_POINT('Ctrl Pts',(16.7523808194749,-19.6969266888527,-20.6671737261315));
#79058=CARTESIAN_POINT('Ctrl Pts',(16.7485503985575,-19.6866424499954,-20.6678277156676));
#79059=CARTESIAN_POINT('Ctrl Pts',(16.7469780574314,-19.6823789764672,-20.668098052724));
#79060=CARTESIAN_POINT('Ctrl Pts',(16.7454194499653,-19.6781104571783,-20.6683679347509));
#79061=CARTESIAN_POINT('',(16.6170007438877,-18.9502252831514,-19.6896814464532));
#79062=CARTESIAN_POINT('Ctrl Pts',(16.7454193204093,-19.6781101023665,-20.4442392291799));
#79063=CARTESIAN_POINT('Ctrl Pts',(16.7951094568911,-19.8141953118298,-20.4346845874371));
#79064=CARTESIAN_POINT('Ctrl Pts',(16.8586919906538,-19.9449671407128,-20.425294583569));
#79065=CARTESIAN_POINT('Ctrl Pts',(16.946440352571,-20.086359051481,-20.4150699224721));
#79066=CARTESIAN_POINT('Ctrl Pts',(16.9579092613415,-20.1042333489413,-20.4137750701033));
#79067=CARTESIAN_POINT('Ctrl Pts',(16.9742421996514,-20.1288647623245,-20.411986945188));
#79068=CARTESIAN_POINT('Ctrl Pts',(16.9788797524813,-20.1357698697497,-20.4114852443744));
#79069=CARTESIAN_POINT('Ctrl Pts',(16.986955549305,-20.1476425809939,-20.4106218243152));
#79070=CARTESIAN_POINT('Ctrl Pts',(16.990374556875,-20.1526230921707,-20.4102593835781));
#79071=CARTESIAN_POINT('Ctrl Pts',(16.9974994304709,-20.1629073596413,-20.409510444408));
#79072=CARTESIAN_POINT('Ctrl Pts',(17.0012083898193,-20.1682089042307,-20.4091240689944));
#79073=CARTESIAN_POINT('Ctrl Pts',(17.0099528057864,-20.1805868716784,-20.4082212208037));
#79074=CARTESIAN_POINT('Ctrl Pts',(17.0150076436039,-20.1876495098593,-20.4077054979974));
#79075=CARTESIAN_POINT('Ctrl Pts',(17.0315678679638,-20.210489219547,-20.4060356641367));
#79076=CARTESIAN_POINT('Ctrl Pts',(17.0432483126324,-20.226138551847,-20.4048883336052));
#79077=CARTESIAN_POINT('Ctrl Pts',(17.1041456281408,-20.3054157636292,-20.3990558829732));
#79078=CARTESIAN_POINT('Ctrl Pts',(17.1567462495226,-20.366366340377,-20.3945073869285));
#79079=CARTESIAN_POINT('Ctrl Pts',(17.3295172146883,-20.544902630157,-20.3807325311516));
#79080=CARTESIAN_POINT('Ctrl Pts',(17.4602838339007,-20.6512793865957,-20.3718906582591));
#79081=CARTESIAN_POINT('Ctrl Pts',(17.6034503023981,-20.7418459276332,-20.3623779523032));
#79082=CARTESIAN_POINT('Ctrl Pts',(17.6046650335289,-20.7426126317282,-20.362297247125));
#79083=CARTESIAN_POINT('Ctrl Pts',(17.6514513430175,-20.7720762866521,-20.359189085107));
#79084=CARTESIAN_POINT('Ctrl Pts',(17.6980966198759,-20.7990225838782,-20.3560999764049));
#79085=CARTESIAN_POINT('Ctrl Pts',(17.7534420180738,-20.8282386341709,-20.3523862265652));
#79086=CARTESIAN_POINT('Ctrl Pts',(17.7611952543453,-20.8322702702407,-20.3518648943258));
#79087=CARTESIAN_POINT('Ctrl Pts',(17.7729670208209,-20.838299220333,-20.3510713889796));
#79088=CARTESIAN_POINT('Ctrl Pts',(17.7769674151895,-20.8403320064167,-20.350801391176));
#79089=CARTESIAN_POINT('Ctrl Pts',(17.7841568778917,-20.8439565923724,-20.3503154890676));
#79090=CARTESIAN_POINT('Ctrl Pts',(17.7873435278836,-20.8455530696404,-20.3500998822104));
#79091=CARTESIAN_POINT('Ctrl Pts',(17.7942733358218,-20.8490029632364,-20.3496304913794));
#79092=CARTESIAN_POINT('Ctrl Pts',(17.7980179022851,-20.850853327131,-20.3493765272743));
#79093=CARTESIAN_POINT('Ctrl Pts',(17.8085434309242,-20.8560157799964,-20.348661803668));
#79094=CARTESIAN_POINT('Ctrl Pts',(17.8153365839922,-20.859302670231,-20.3481995228626));
#79095=CARTESIAN_POINT('Ctrl Pts',(17.8558881851492,-20.8786568022995,-20.3454346552672));
#79096=CARTESIAN_POINT('Ctrl Pts',(17.8900476785133,-20.8938627334018,-20.343083932858));
#79097=CARTESIAN_POINT('Ctrl Pts',(18.0034024770103,-20.9407662663708,-20.3352546161963));
#79098=CARTESIAN_POINT('Ctrl Pts',(18.0841095782876,-20.9685823989571,-20.3296382171641));
#79099=CARTESIAN_POINT('Ctrl Pts',(18.3376598380881,-21.0391643154831,-20.3122512383248));
#79100=CARTESIAN_POINT('Ctrl Pts',(18.5144189555838,-21.0650899138362,-20.3005605532114));
#79101=CARTESIAN_POINT('Ctrl Pts',(18.7151580919771,-21.0690389382767,-20.2882046024328));
#79102=CARTESIAN_POINT('Ctrl Pts',(18.7379610600611,-21.0691190938378,-20.2868128522382));
#79103=CARTESIAN_POINT('Ctrl Pts',(18.770275709497,-21.0687105625804,-20.2848566432985));
#79104=CARTESIAN_POINT('Ctrl Pts',(18.7797890236273,-21.0685261403483,-20.2842827139751));
#79105=CARTESIAN_POINT('Ctrl Pts',(18.7952600020699,-21.0681218649598,-20.283352488968));
#79106=CARTESIAN_POINT('Ctrl Pts',(18.8012184723263,-21.0679409758598,-20.2829949773939));
#79107=CARTESIAN_POINT('Ctrl Pts',(18.8137017416473,-21.0675092216074,-20.2822475242478));
#79108=CARTESIAN_POINT('Ctrl Pts',(18.8202263128847,-21.0672533320544,-20.2818577441247));
#79109=CARTESIAN_POINT('Ctrl Pts',(18.8357680782531,-21.0665717643682,-20.2809313396686));
#79110=CARTESIAN_POINT('Ctrl Pts',(18.8447839860368,-21.0661185871886,-20.2803955826443));
#79111=CARTESIAN_POINT('Ctrl Pts',(18.875256604488,-21.0643914346441,-20.2785901930243));
#79112=CARTESIAN_POINT('Ctrl Pts',(18.8966971650678,-21.0628483327842,-20.2773289945289));
#79113=CARTESIAN_POINT('Ctrl Pts',(19.0968825238194,-21.0453724124202,-20.2656291356277));
#79114=CARTESIAN_POINT('Ctrl Pts',(19.2729416028154,-21.0071011457111,-20.2559872354047));
#79115=CARTESIAN_POINT('Ctrl Pts',(19.5556343147672,-20.9067700395057,-20.2396620219451));
#79116=CARTESIAN_POINT('Ctrl Pts',(19.6655284762268,-20.8568504082491,-20.2330511826679));
#79117=CARTESIAN_POINT('Ctrl Pts',(19.7788432733866,-20.7932174527959,-20.2253489775442));
#79118=CARTESIAN_POINT('Ctrl Pts',(19.7870915475381,-20.7885122812894,-20.2247829502586));
#79119=CARTESIAN_POINT('Ctrl Pts',(19.7992711765382,-20.7814554662475,-20.2239387152781));
#79120=CARTESIAN_POINT('Ctrl Pts',(19.8032271336972,-20.7791462224482,-20.223663179313));
#79121=CARTESIAN_POINT('Ctrl Pts',(19.810254393918,-20.7750135044969,-20.22317130045));
#79122=CARTESIAN_POINT('Ctrl Pts',(19.8133286074333,-20.7731950787742,-20.2229552864762));
#79123=CARTESIAN_POINT('Ctrl Pts',(19.8199306225379,-20.7692673378157,-20.222489578866));
#79124=CARTESIAN_POINT('Ctrl Pts',(19.8234568357825,-20.7671555570695,-20.2222397295855));
#79125=CARTESIAN_POINT('Ctrl Pts',(19.8331790941365,-20.7612945495431,-20.2215478399339));
#79126=CARTESIAN_POINT('Ctrl Pts',(19.8393620165736,-20.7575238178486,-20.2211044277628));
#79127=CARTESIAN_POINT('Ctrl Pts',(19.8732234723351,-20.7366338706383,-20.2186578162648));
#79128=CARTESIAN_POINT('Ctrl Pts',(19.9005221458512,-20.7189108596778,-20.2166182569852));
#79129=CARTESIAN_POINT('Ctrl Pts',(20.0617807904764,-20.6088515790043,-20.2042120968778));
#79130=CARTESIAN_POINT('Ctrl Pts',(20.185137890794,-20.5019541075133,-20.1932557254062));
#79131=CARTESIAN_POINT('Ctrl Pts',(20.3739364858185,-20.2958532227758,-20.1749987219105));
#79132=CARTESIAN_POINT('Ctrl Pts',(20.4455836971107,-20.2033281804784,-20.1675581068973));
#79133=CARTESIAN_POINT('Ctrl Pts',(20.5170242806521,-20.0933665485799,-20.1595512610459));
#79134=CARTESIAN_POINT('Ctrl Pts',(20.5246877590987,-20.0813053390216,-20.1586832888641));
#79135=CARTESIAN_POINT('Ctrl Pts',(20.5366902189829,-20.0619857894196,-20.1573089857889));
#79136=CARTESIAN_POINT('Ctrl Pts',(20.5411087459664,-20.0547776121328,-20.1567997268503));
#79137=CARTESIAN_POINT('Ctrl Pts',(20.548825354215,-20.0420181754053,-20.1559043513171));
#79138=CARTESIAN_POINT('Ctrl Pts',(20.5521414195464,-20.0364779707204,-20.1555175785997));
#79139=CARTESIAN_POINT('Ctrl Pts',(20.5589476838088,-20.024987667407,-20.1547195114838));
#79140=CARTESIAN_POINT('Ctrl Pts',(20.5624342550248,-20.0190355007357,-20.1543083524671));
#79141=CARTESIAN_POINT('Ctrl Pts',(20.5713091281875,-20.003713361264,-20.1532556439074));
#79142=CARTESIAN_POINT('Ctrl Pts',(20.5766549181833,-19.9943188983395,-20.1526156356688));
#79143=CARTESIAN_POINT('Ctrl Pts',(20.5986660915895,-19.9549387880268,-20.1499549682845));
#79144=CARTESIAN_POINT('Ctrl Pts',(20.6146738833644,-19.9245902460364,-20.1479578380001));
#79145=CARTESIAN_POINT('Ctrl Pts',(20.6544542961342,-19.8445137945479,-20.1428137515898));
#79146=CARTESIAN_POINT('Ctrl Pts',(20.677035763032,-19.7942222070087,-20.1397061847616));
#79147=CARTESIAN_POINT('Ctrl Pts',(20.738492048994,-19.641679115766,-20.1305617623255));
#79148=CARTESIAN_POINT('Ctrl Pts',(20.7714353569377,-19.5372381627218,-20.1246736362835));
#79149=CARTESIAN_POINT('Ctrl Pts',(20.8065062231099,-19.3861648461232,-20.1162298524835));
#79150=CARTESIAN_POINT('Ctrl Pts',(20.8154024978397,-19.3412872499354,-20.1137288737193));
#79151=CARTESIAN_POINT('Ctrl Pts',(20.8265388435982,-19.2736961695852,-20.1099303523099));
#79152=CARTESIAN_POINT('Ctrl Pts',(20.8298770511543,-19.2511764901954,-20.1086595135307));
#79153=CARTESIAN_POINT('Ctrl Pts',(20.8329763866112,-19.2276592897455,-20.1073230258424));
#79154=CARTESIAN_POINT('Ctrl Pts',(20.8331007664771,-19.2267105526645,-20.1072690930572));
#79155=CARTESIAN_POINT('Ctrl Pts',(20.835414482207,-19.2089688153357,-20.1062602282928));
#79156=CARTESIAN_POINT('Ctrl Pts',(20.8374028260142,-19.192150623561,-20.105298830823));
#79157=CARTESIAN_POINT('Ctrl Pts',(20.8428628448425,-19.1406780920217,-20.1023362274941));
#79158=CARTESIAN_POINT('Ctrl Pts',(20.8456811406815,-19.1059622224045,-20.1003101554433));
#79159=CARTESIAN_POINT('Ctrl Pts',(20.8480368528763,-19.0641892209831,-20.0978219876125));
#79160=CARTESIAN_POINT('Ctrl Pts',(20.8483970894526,-19.0571816601472,-20.0974028934515));
#79161=CARTESIAN_POINT('Ctrl Pts',(20.8489299572372,-19.0457032225027,-20.0967134499008));
#79162=CARTESIAN_POINT('Ctrl Pts',(20.8491232672893,-19.0412332967747,-20.0964442314703));
#79163=CARTESIAN_POINT('Ctrl Pts',(20.8494450792549,-19.0332023054611,-20.0959591591568));
#79164=CARTESIAN_POINT('Ctrl Pts',(20.8495787611597,-19.0296415016763,-20.0957435982898));
#79165=CARTESIAN_POINT('Ctrl Pts',(20.8498499661962,-19.0218959990634,-20.0952736348228));
#79166=CARTESIAN_POINT('Ctrl Pts',(20.8499840635673,-19.0177112788362,-20.0950190484162));
#79167=CARTESIAN_POINT('Ctrl Pts',(20.8503264209045,-19.00593639317,-20.094300849607));
#79168=CARTESIAN_POINT('Ctrl Pts',(20.8505062579293,-18.9983455549318,-20.0938356925313));
#79169=CARTESIAN_POINT('Ctrl Pts',(20.8513445290428,-18.9525613666721,-20.0910177338244));
#79170=CARTESIAN_POINT('Ctrl Pts',(20.8510099044863,-18.9143594262355,-20.0886146656814));
#79171=CARTESIAN_POINT('Ctrl Pts',(20.8464731240225,-18.7877501482996,-20.0805234784596));
#79172=CARTESIAN_POINT('Ctrl Pts',(20.8377617606703,-18.6996010815258,-20.0746880681203));
#79173=CARTESIAN_POINT('Ctrl Pts',(20.7957454093421,-18.4411791377453,-20.0573881260028));
#79174=CARTESIAN_POINT('Ctrl Pts',(20.7470176745464,-18.2741249616737,-20.0460171671181));
#79175=CARTESIAN_POINT('Ctrl Pts',(20.6693002344558,-18.0936075860013,-20.0339182115918));
#79176=CARTESIAN_POINT('Ctrl Pts',(20.6598010428807,-18.0725030165807,-20.0325053599962));
#79177=CARTESIAN_POINT('Ctrl Pts',(20.6458865243582,-18.0428957593003,-20.0305249464703));
#79178=CARTESIAN_POINT('Ctrl Pts',(20.6417568959298,-18.0342613480849,-20.0299475930393));
#79179=CARTESIAN_POINT('Ctrl Pts',(20.6349559097492,-18.0202858347727,-20.0290133369963));
#79180=CARTESIAN_POINT('Ctrl Pts',(20.6323202933435,-18.0149275793667,-20.0286551974926));
#79181=CARTESIAN_POINT('Ctrl Pts',(20.6267592450396,-18.0037416180122,-20.0279076308146));
#79182=CARTESIAN_POINT('Ctrl Pts',(20.623829484195,-17.9979161248468,-20.0275183598308));
#79183=CARTESIAN_POINT('Ctrl Pts',(20.6168018773392,-17.9841019165005,-20.0265953404202));
#79184=CARTESIAN_POINT('Ctrl Pts',(20.6126800130813,-17.976125509307,-20.0260624423581));
#79185=CARTESIAN_POINT('Ctrl Pts',(20.5986527563105,-17.9493989976437,-20.0242768600043));
#79186=CARTESIAN_POINT('Ctrl Pts',(20.5885162192826,-17.9307711754583,-20.0230323561497));
#79187=CARTESIAN_POINT('Ctrl Pts',(20.5320177019306,-17.8305607171013,-20.016332306278));
#79188=CARTESIAN_POINT('Ctrl Pts',(20.4805481446169,-17.7519723921545,-20.0110657388705));
#79189=CARTESIAN_POINT('Ctrl Pts',(20.3279480334004,-17.549690934078,-19.9971172333309));
#79190=CARTESIAN_POINT('Ctrl Pts',(20.2177889895693,-17.4336115924511,-19.9886941392892));
#79191=CARTESIAN_POINT('Ctrl Pts',(20.0890806216629,-17.3254948106074,-19.9791997111178));
#79192=CARTESIAN_POINT('Ctrl Pts',(20.0824772395814,-17.3200160070786,-19.9787133535409));
#79193=CARTESIAN_POINT('Ctrl Pts',(20.0445540837438,-17.2889386032625,-19.9759233255696));
#79194=CARTESIAN_POINT('Ctrl Pts',(20.0125411923671,-17.2642034608607,-19.9735802302566));
#79195=CARTESIAN_POINT('Ctrl Pts',(19.9738960313434,-17.23607432669,-19.9707399083838));
#79196=CARTESIAN_POINT('Ctrl Pts',(19.9679277020679,-17.2317774831808,-19.9703009269887));
#79197=CARTESIAN_POINT('Ctrl Pts',(19.9582089751464,-17.2248571766077,-19.9695853584113));
#79198=CARTESIAN_POINT('Ctrl Pts',(19.9544721870562,-17.2222145835555,-19.9693100511876));
#79199=CARTESIAN_POINT('Ctrl Pts',(19.9478042275556,-17.2175314783284,-19.968818421559));
#79200=CARTESIAN_POINT('Ctrl Pts',(19.9448764332441,-17.2154862457548,-19.9686024267764));
#79201=CARTESIAN_POINT('Ctrl Pts',(19.938565837533,-17.2111016518852,-19.9681365787778));
#79202=CARTESIAN_POINT('Ctrl Pts',(19.9351814397367,-17.2087647710112,-19.9678865689566));
#79203=CARTESIAN_POINT('Ctrl Pts',(19.9258091288351,-17.2023335691307,-19.9671937942238));
#79204=CARTESIAN_POINT('Ctrl Pts',(19.9198070145729,-17.1982601847573,-19.9667496518529));
#79205=CARTESIAN_POINT('Ctrl Pts',(19.886617890084,-17.17598438511,-19.9642916133847));
#79206=CARTESIAN_POINT('Ctrl Pts',(19.859034239654,-17.1583843357344,-19.962240964186));
#79207=CARTESIAN_POINT('Ctrl Pts',(19.6920336853364,-17.0571957160218,-19.9498310162141));
#79208=CARTESIAN_POINT('Ctrl Pts',(19.5437766951488,-16.9892535887587,-19.9388847359663));
#79209=CARTESIAN_POINT('Ctrl Pts',(19.2781805894784,-16.9028076619477,-19.9206407205647));
#79210=CARTESIAN_POINT('Ctrl Pts',(19.1643411956418,-16.8759132956713,-19.913203361494));
#79211=CARTESIAN_POINT('Ctrl Pts',(19.034717565091,-16.8564184311949,-19.9051995451461));
#79212=CARTESIAN_POINT('Ctrl Pts',(19.0205664076742,-16.8544364431137,-19.9043316120189));
#79213=CARTESIAN_POINT('Ctrl Pts',(18.9980119584396,-16.8515100187934,-19.9029573584115));
#79214=CARTESIAN_POINT('Ctrl Pts',(18.9896213922512,-16.8504724169283,-19.9024481102261));
#79215=CARTESIAN_POINT('Ctrl Pts',(18.9748122342812,-16.8487310783971,-19.9015527466365));
#79216=CARTESIAN_POINT('Ctrl Pts',(18.9683962590684,-16.8480063964148,-19.9011659751714));
#79217=CARTESIAN_POINT('Ctrl Pts',(18.9551189912645,-16.8465682210066,-19.9003679039678));
#79218=CARTESIAN_POINT('Ctrl Pts',(18.948257318076,-16.8458588870458,-19.8999567396444));
#79219=CARTESIAN_POINT('Ctrl Pts',(18.9306352119817,-16.8441241904971,-19.8989040036792));
#79220=CARTESIAN_POINT('Ctrl Pts',(18.9198700873584,-16.8431476694507,-19.898263973491));
#79221=CARTESIAN_POINT('Ctrl Pts',(18.8749070161365,-16.8394159720983,-19.8956030992208));
#79222=CARTESIAN_POINT('Ctrl Pts',(18.840650991737,-16.8374097737959,-19.8936057886063));
#79223=CARTESIAN_POINT('Ctrl Pts',(18.7512799517122,-16.8343532529321,-19.8884611346919));
#79224=CARTESIAN_POINT('Ctrl Pts',(18.6961450163041,-16.834620962625,-19.8853531919853));
#79225=CARTESIAN_POINT('Ctrl Pts',(18.4578825206337,-16.8450889183847,-19.8720922416621));
#79226=CARTESIAN_POINT('Ctrl Pts',(18.2765290384972,-16.8769038756254,-19.8625001067257));
#79227=CARTESIAN_POINT('Ctrl Pts',(18.0574431867915,-16.9454864106654,-19.8495086414657));
#79228=CARTESIAN_POINT('Ctrl Pts',(18.0137951913747,-16.9607365193418,-19.8468424005504));
#79229=CARTESIAN_POINT('Ctrl Pts',(17.9635506949731,-16.9801593949427,-19.8436435510397));
#79230=CARTESIAN_POINT('Ctrl Pts',(17.9564315646845,-16.9829558593639,-19.8431872202555));
#79231=CARTESIAN_POINT('Ctrl Pts',(17.9450411793493,-16.9875015190664,-19.8424519074684));
#79232=CARTESIAN_POINT('Ctrl Pts',(17.9407601441824,-16.9892262401154,-19.8421743598098));
#79233=CARTESIAN_POINT('Ctrl Pts',(17.9331647342377,-16.9923151469594,-19.8416797724876));
#79234=CARTESIAN_POINT('Ctrl Pts',(17.9298481455986,-16.9936737654281,-19.841463070751));
#79235=CARTESIAN_POINT('Ctrl Pts',(17.9227996537634,-16.9965820584099,-19.8410009421983));
#79236=CARTESIAN_POINT('Ctrl Pts',(17.919068790636,-16.9981339730167,-19.840755385955));
#79237=CARTESIAN_POINT('Ctrl Pts',(17.9090820094276,-17.00232172058,-19.8400955893012));
#79238=CARTESIAN_POINT('Ctrl Pts',(17.9028343500244,-17.0049769534421,-19.8396801983692));
#79239=CARTESIAN_POINT('Ctrl Pts',(17.8719118144841,-17.0182948762989,-19.8376115761724));
#79240=CARTESIAN_POINT('Ctrl Pts',(17.8474300203297,-17.0293962812278,-19.8359337265203));
#79241=CARTESIAN_POINT('Ctrl Pts',(17.777230875773,-17.062854325332,-19.8310195190076));
#79242=CARTESIAN_POINT('Ctrl Pts',(17.7321014556109,-17.0863963038991,-19.8277316425662));
#79243=CARTESIAN_POINT('Ctrl Pts',(17.6012698609584,-17.1607620478373,-19.8178997079442));
#79244=CARTESIAN_POINT('Ctrl Pts',(17.5182551517247,-17.2160347110697,-19.8112703400073));
#79245=CARTESIAN_POINT('Ctrl Pts',(17.4275637978787,-17.2861252294552,-19.8037403397405));
#79246=CARTESIAN_POINT('Ctrl Pts',(17.4157851062505,-17.2954301089221,-19.802756214046));
#79247=CARTESIAN_POINT('Ctrl Pts',(17.3105976467623,-17.3803579882302,-19.7939148841377));
#79248=CARTESIAN_POINT('Ctrl Pts',(17.2236759054821,-17.4636914070113,-19.7862491314523));
#79249=CARTESIAN_POINT('Ctrl Pts',(17.133907704203,-17.5657674731961,-19.7779486627357));
#79250=CARTESIAN_POINT('Ctrl Pts',(17.1236610246714,-17.5776840323712,-19.7769945202234));
#79251=CARTESIAN_POINT('Ctrl Pts',(17.1083597659514,-17.5958850239516,-19.7755591886708));
#79252=CARTESIAN_POINT('Ctrl Pts',(17.103207002873,-17.6020858537861,-19.7750739796163));
#79253=CARTESIAN_POINT('Ctrl Pts',(17.0940373121159,-17.6132497819579,-19.7742071116631));
#79254=CARTESIAN_POINT('Ctrl Pts',(17.0900071984328,-17.6182018766924,-19.7738249196995));
#79255=CARTESIAN_POINT('Ctrl Pts',(17.0815036577164,-17.6287478924441,-19.7730158948805));
#79256=CARTESIAN_POINT('Ctrl Pts',(17.0770360844197,-17.6343464469702,-19.7725893005581));
#79257=CARTESIAN_POINT('Ctrl Pts',(17.0651573365794,-17.6493882919641,-19.7714507848237));
#79258=CARTESIAN_POINT('Ctrl Pts',(17.0577978546972,-17.6588722127342,-19.770740926658));
#79259=CARTESIAN_POINT('Ctrl Pts',(17.0223745414901,-17.7053316367734,-19.7673013352193));
#79260=CARTESIAN_POINT('Ctrl Pts',(16.9954500887626,-17.7431623789647,-19.7646164247055));
#79261=CARTESIAN_POINT('Ctrl Pts',(16.919785290694,-17.8572405882314,-19.7568180538405));
#79262=CARTESIAN_POINT('Ctrl Pts',(16.8746620068182,-17.9357631156808,-19.75182947175));
#79263=CARTESIAN_POINT('Ctrl Pts',(16.8015554844187,-18.0842571027667,-19.7428030122621));
#79264=CARTESIAN_POINT('Ctrl Pts',(16.772015276171,-18.1532914773746,-19.7387531925283));
#79265=CARTESIAN_POINT('Ctrl Pts',(16.710891428836,-18.3201317462362,-19.7290386440713));
#79266=CARTESIAN_POINT('Ctrl Pts',(16.6826415341211,-18.4189441223155,-19.7233418111299));
#79267=CARTESIAN_POINT('Ctrl Pts',(16.6596911929394,-18.5288855123653,-19.7166879680927));
#79268=CARTESIAN_POINT('Ctrl Pts',(16.6577762683325,-18.5383843514854,-19.7161105270604));
#79269=CARTESIAN_POINT('Ctrl Pts',(16.6550450479744,-18.5524294323368,-19.7152525031138));
#79270=CARTESIAN_POINT('Ctrl Pts',(16.6541782809238,-18.5569658913124,-19.7149747201565));
#79271=CARTESIAN_POINT('Ctrl Pts',(16.6526668272638,-18.5650193685107,-19.7144803720146));
#79272=CARTESIAN_POINT('Ctrl Pts',(16.6520161987248,-18.5685352218286,-19.7142641484818));
#79273=CARTESIAN_POINT('Ctrl Pts',(16.650641182941,-18.5760721707847,-19.7137997354823));
#79274=CARTESIAN_POINT('Ctrl Pts',(16.6499195393132,-18.580093659469,-19.7135513995312));
#79275=CARTESIAN_POINT('Ctrl Pts',(16.6484624965497,-18.5883507147415,-19.7130404375919));
#79276=CARTESIAN_POINT('Ctrl Pts',(16.647728348886,-18.5925864805177,-19.7127777434399));
#79277=CARTESIAN_POINT('Ctrl Pts',(16.6459030758296,-18.603311687976,-19.7121111777086));
#79278=CARTESIAN_POINT('Ctrl Pts',(16.6448293063746,-18.6098039830409,-19.7117063815082));
#79279=CARTESIAN_POINT('Ctrl Pts',(16.6260483532597,-18.7267427401032,-19.7043930655705));
#79280=CARTESIAN_POINT('Ctrl Pts',(16.6170944882044,-18.8384008820488,-19.6970632328612));
#79281=CARTESIAN_POINT('Ctrl Pts',(16.6170007438877,-18.9502252831514,-19.6896814464532));
#79282=CARTESIAN_POINT('Ctrl Pts',(16.6170007453285,-18.9502235652229,-19.6896815598576));
#79283=CARTESIAN_POINT('Ctrl Pts',(16.6169157215329,-19.0515474721257,-19.6829929357409));
#79284=CARTESIAN_POINT('Ctrl Pts',(16.624105218519,-19.1527558515676,-19.676279183763));
#79285=CARTESIAN_POINT('Ctrl Pts',(16.6510570136956,-19.34034580853,-19.6640088596727));
#79286=CARTESIAN_POINT('Ctrl Pts',(16.6690385649789,-19.4267648125115,-19.6584257671682));
#79287=CARTESIAN_POINT('Ctrl Pts',(16.6977854267898,-19.5316033194997,-19.6517542931015));
#79288=CARTESIAN_POINT('Ctrl Pts',(16.7034973725127,-19.5513070351543,-19.6505046733498));
#79289=CARTESIAN_POINT('Ctrl Pts',(16.7120850741006,-19.5793974178702,-19.6487287240108));
#79290=CARTESIAN_POINT('Ctrl Pts',(16.7147283676524,-19.587853415537,-19.6481948376127));
#79291=CARTESIAN_POINT('Ctrl Pts',(16.7194027738261,-19.6024838660219,-19.647272300583));
#79292=CARTESIAN_POINT('Ctrl Pts',(16.7214093686994,-19.6086659698244,-19.6468828508525));
#79293=CARTESIAN_POINT('Ctrl Pts',(16.7253223050648,-19.6205348830199,-19.6461358268466));
#79294=CARTESIAN_POINT('Ctrl Pts',(16.7272244027105,-19.6262230159287,-19.6457781171379));
#79295=CARTESIAN_POINT('Ctrl Pts',(16.7322706374349,-19.641102991212,-19.6448431009333));
#79296=CARTESIAN_POINT('Ctrl Pts',(16.7354539394052,-19.6502814775665,-19.6442670940895));
#79297=CARTESIAN_POINT('Ctrl Pts',(16.7409108787423,-19.6656725528941,-19.6433023316371));
#79298=CARTESIAN_POINT('Ctrl Pts',(16.743150603721,-19.671896824708,-19.6429124843661));
#79299=CARTESIAN_POINT('Ctrl Pts',(16.7454194498907,-19.678110456974,-19.6425235871583));
#79300=CARTESIAN_POINT('Origin',(18.734,-18.952,0.));
#79301=CARTESIAN_POINT('',(16.7454194032426,-19.6781103292199,-18.8452753983371));
#79302=CARTESIAN_POINT('',(16.7454194499637,-19.6781104571739,-19.0663245191576));
#79303=CARTESIAN_POINT('',(16.7454194499637,-19.6781104571739,0.));
#79304=CARTESIAN_POINT('',(16.6180378855072,-18.9538841874204,-19.1109437209775));
#79305=CARTESIAN_POINT('Ctrl Pts',(16.7454194499637,-19.6781104571739,-19.0663245191576));
#79306=CARTESIAN_POINT('Ctrl Pts',(16.7290739263666,-19.6333453804777,-19.0692018282141));
#79307=CARTESIAN_POINT('Ctrl Pts',(16.7142587319683,-19.5880774621226,-19.0720791372705));
#79308=CARTESIAN_POINT('Ctrl Pts',(16.7009992479656,-19.5424209872857,-19.074956446327));
#79309=CARTESIAN_POINT('Ctrl Pts',(16.6758066766558,-19.4556752287146,-19.0804232362541));
#79310=CARTESIAN_POINT('Ctrl Pts',(16.6561521069708,-19.367253508475,-19.0858900261813));
#79311=CARTESIAN_POINT('Ctrl Pts',(16.6422180861824,-19.2777873923673,-19.0913568161084));
#79312=CARTESIAN_POINT('Ctrl Pts',(16.6285119268914,-19.1897843057392,-19.0967342082258));
#79313=CARTESIAN_POINT('Ctrl Pts',(16.6203407792448,-19.1007706087263,-19.1021116003432));
#79314=CARTESIAN_POINT('Ctrl Pts',(16.6178326248366,-19.0113686810859,-19.1074889924606));
#79315=CARTESIAN_POINT('Ctrl Pts',(16.6172955000017,-18.9922231310909,-19.1086405686329));
#79316=CARTESIAN_POINT('Ctrl Pts',(16.6170179137274,-18.9730598582114,-19.1097921448052));
#79317=CARTESIAN_POINT('Ctrl Pts',(16.6170008393112,-18.9538851108724,-19.1109437209775));
#79318=CARTESIAN_POINT('Ctrl Pts',(16.6180378855072,-18.9538841874204,-19.1109437209775));
#79319=CARTESIAN_POINT('Ctrl Pts',(16.622366738429,-18.4480050085671,-19.1413398983212));
#79320=CARTESIAN_POINT('Ctrl Pts',(17.0578064022828,-17.2299118723797,-19.2141280112252));
#79321=CARTESIAN_POINT('Ctrl Pts',(19.0938031787897,-16.4747288712945,-19.3293080596899));
#79322=CARTESIAN_POINT('Ctrl Pts',(21.0117476238401,-17.913637640173,-19.4564838663712));
#79323=CARTESIAN_POINT('Ctrl Pts',(20.8399999988754,-20.3051794704029,-19.5836596730529));
#79324=CARTESIAN_POINT('Ctrl Pts',(18.7361280843893,-21.4552630390637,-19.7108354797341));
#79325=CARTESIAN_POINT('Ctrl Pts',(17.1750895211376,-20.6053639705819,-19.8051103626019));
#79326=CARTESIAN_POINT('Ctrl Pts',(16.7978195176575,-19.8268833696163,-19.856993309909));
#79327=CARTESIAN_POINT('Ctrl Pts',(16.7452305273115,-19.6781794125984,-19.8664843216556));
#79328=CARTESIAN_POINT('Ctrl Pts',(16.7454194498907,-19.678110456974,-19.6425235871583));
#79329=CARTESIAN_POINT('Ctrl Pts',(16.7513832064613,-19.6944432479537,-19.6415013546644));
#79330=CARTESIAN_POINT('Ctrl Pts',(16.7575481680138,-19.7107025283047,-19.6404856934997));
#79331=CARTESIAN_POINT('Ctrl Pts',(16.8191736666767,-19.8673808173857,-19.6307122755094));
#79332=CARTESIAN_POINT('Ctrl Pts',(16.8893050312533,-20.0015661897086,-19.6224919227194));
#79333=CARTESIAN_POINT('Ctrl Pts',(17.0102352499799,-20.1827695245077,-19.6106616261116));
#79334=CARTESIAN_POINT('Ctrl Pts',(17.0499589213118,-20.2365869578084,-19.6070351305032));
#79335=CARTESIAN_POINT('Ctrl Pts',(17.1263126030287,-20.3303892442845,-19.6003481701723));
#79336=CARTESIAN_POINT('Ctrl Pts',(17.1620578397331,-20.3710182217699,-19.5973138498835));
#79337=CARTESIAN_POINT('Ctrl Pts',(17.2185936143475,-20.4305180581435,-19.5925772640953));
#79338=CARTESIAN_POINT('Ctrl Pts',(17.2382695806024,-20.4504200023401,-19.5909393363386));
#79339=CARTESIAN_POINT('Ctrl Pts',(17.2632160887945,-20.474672014578,-19.5888664616147));
#79340=CARTESIAN_POINT('Ctrl Pts',(17.2681218468328,-20.4793953694554,-19.5884590057323));
#79341=CARTESIAN_POINT('Ctrl Pts',(17.2760082684952,-20.4869155732619,-19.587804099952));
#79342=CARTESIAN_POINT('Ctrl Pts',(17.2789744377563,-20.4897276477795,-19.5875578083018));
#79343=CARTESIAN_POINT('Ctrl Pts',(17.2845504956219,-20.4949834469785,-19.5870948134674));
#79344=CARTESIAN_POINT('Ctrl Pts',(17.2871584375725,-20.4974291559132,-19.586878267291));
#79345=CARTESIAN_POINT('Ctrl Pts',(17.2931476521016,-20.5030173499238,-19.5863809687617));
#79346=CARTESIAN_POINT('Ctrl Pts',(17.2965330058392,-20.5061553808984,-19.5860998827092));
#79347=CARTESIAN_POINT('Ctrl Pts',(17.3054342628809,-20.5143523781155,-19.5853608968982));
#79348=CARTESIAN_POINT('Ctrl Pts',(17.3109667232938,-20.5193931568867,-19.5849016758516));
#79349=CARTESIAN_POINT('Ctrl Pts',(17.3483958362069,-20.5531343530628,-19.5817961650597));
#79350=CARTESIAN_POINT('Ctrl Pts',(17.3811296666267,-20.5808865522599,-19.5790866178343));
#79351=CARTESIAN_POINT('Ctrl Pts',(17.4212483212683,-20.6128559665986,-19.5757959124704));
#79352=CARTESIAN_POINT('Ctrl Pts',(17.4278463901912,-20.6180498960387,-19.5752556461949));
#79353=CARTESIAN_POINT('Ctrl Pts',(17.4457534187519,-20.6319743625904,-19.5737922505113));
#79354=CARTESIAN_POINT('Ctrl Pts',(17.4571200312392,-20.6406298127629,-19.572866419495));
#79355=CARTESIAN_POINT('Ctrl Pts',(17.5768592650271,-20.7299086070912,-19.5631519091738));
#79356=CARTESIAN_POINT('Ctrl Pts',(17.6926242410796,-20.8000996500337,-19.5541120302114));
#79357=CARTESIAN_POINT('Ctrl Pts',(17.9141593465285,-20.9069537602988,-19.5380905046534));
#79358=CARTESIAN_POINT('Ctrl Pts',(18.0176687647134,-20.9472090654657,-19.5310500916392));
#79359=CARTESIAN_POINT('Ctrl Pts',(18.1382376049595,-20.9834972954317,-19.5233698644076));
#79360=CARTESIAN_POINT('Ctrl Pts',(18.1526499363599,-20.9876684932426,-19.5224597225658));
#79361=CARTESIAN_POINT('Ctrl Pts',(18.1746298980515,-20.9937774305612,-19.5210834355425));
#79362=CARTESIAN_POINT('Ctrl Pts',(18.182165697115,-20.9958270209614,-19.5206136642382));
#79363=CARTESIAN_POINT('Ctrl Pts',(18.1958625178662,-20.9994710124786,-19.5197635505702));
#79364=CARTESIAN_POINT('Ctrl Pts',(18.2020196882585,-21.0010794142507,-19.5193827581294));
#79365=CARTESIAN_POINT('Ctrl Pts',(18.2152898241597,-21.0044820498446,-19.5185649500938));
#79366=CARTESIAN_POINT('Ctrl Pts',(18.2224050678729,-21.0062671294049,-19.5181282347316));
#79367=CARTESIAN_POINT('Ctrl Pts',(18.2416306582839,-21.0109843819199,-19.5169529332033));
#79368=CARTESIAN_POINT('Ctrl Pts',(18.2537579676296,-21.0138467096242,-19.5162166014125));
#79369=CARTESIAN_POINT('Ctrl Pts',(18.3117601982119,-21.0269970716835,-19.5127180538857));
#79370=CARTESIAN_POINT('Ctrl Pts',(18.357946135052,-21.0358625850952,-19.5100015925458));
#79371=CARTESIAN_POINT('Ctrl Pts',(18.4449512248838,-21.0495761606526,-19.5049896018816));
#79372=CARTESIAN_POINT('Ctrl Pts',(18.4856895137337,-21.0547879351184,-19.5026853727095));
#79373=CARTESIAN_POINT('Ctrl Pts',(18.6850377352986,-21.0744165262435,-19.4915595754524));
#79374=CARTESIAN_POINT('Ctrl Pts',(18.8447634385835,-21.0720887461264,-19.4831458930242));
#79375=CARTESIAN_POINT('Ctrl Pts',(19.0484598722091,-21.0460227443856,-19.4717142623738));
#79376=CARTESIAN_POINT('Ctrl Pts',(19.0940027330479,-21.038675287285,-19.4691089522826));
#79377=CARTESIAN_POINT('Ctrl Pts',(19.1557108640872,-21.0266396459103,-19.4654681083536));
#79378=CARTESIAN_POINT('Ctrl Pts',(19.1721163181589,-21.0232372556315,-19.4644893620884));
#79379=CARTESIAN_POINT('Ctrl Pts',(19.2001422140399,-21.0170770048535,-19.4627961245304));
#79380=CARTESIAN_POINT('Ctrl Pts',(19.2117830979068,-21.0144148215717,-19.4620865079337));
#79381=CARTESIAN_POINT('Ctrl Pts',(19.2282926041553,-21.0104919492343,-19.4610703168165));
#79382=CARTESIAN_POINT('Ctrl Pts',(19.2331804614697,-21.0093121176148,-19.4607682361835));
#79383=CARTESIAN_POINT('Ctrl Pts',(19.2415939745128,-21.0072495144299,-19.4602460790663));
#79384=CARTESIAN_POINT('Ctrl Pts',(19.2451216828042,-21.0063750472448,-19.4600264801571));
#79385=CARTESIAN_POINT('Ctrl Pts',(19.2519551409747,-21.0046624423578,-19.459599785814));
#79386=CARTESIAN_POINT('Ctrl Pts',(19.2552611250853,-21.0038253993509,-19.4593927596644));
#79387=CARTESIAN_POINT('Ctrl Pts',(19.264170918735,-21.0015466031443,-19.4588332379587));
#79388=CARTESIAN_POINT('Ctrl Pts',(19.269770815251,-21.0000898694273,-19.4584798895516));
#79389=CARTESIAN_POINT('Ctrl Pts',(19.2905078471284,-20.9946045577946,-19.4571653371271));
#79390=CARTESIAN_POINT('Ctrl Pts',(19.3056056722854,-20.9904310843758,-19.4561962625258));
#79391=CARTESIAN_POINT('Ctrl Pts',(19.449767543781,-20.9488531318853,-19.4468369344059));
#79392=CARTESIAN_POINT('Ctrl Pts',(19.5750295841489,-20.8994107506389,-19.4379069223211));
#79393=CARTESIAN_POINT('Ctrl Pts',(19.837816238959,-20.7655754525965,-19.4184305523235));
#79394=CARTESIAN_POINT('Ctrl Pts',(19.9721561617023,-20.6766606795245,-19.4079968559008));
#79395=CARTESIAN_POINT('Ctrl Pts',(20.1094539179999,-20.5613984819543,-19.3970168073795));
#79396=CARTESIAN_POINT('Ctrl Pts',(20.1235816983893,-20.5492162322996,-19.3958819751655));
#79397=CARTESIAN_POINT('Ctrl Pts',(20.1439297388161,-20.5311959419061,-19.3942396949984));
#79398=CARTESIAN_POINT('Ctrl Pts',(20.1502783601182,-20.5255047827425,-19.3937261681634));
#79399=CARTESIAN_POINT('Ctrl Pts',(20.1613653292252,-20.5154445154962,-19.3928272999184));
#79400=CARTESIAN_POINT('Ctrl Pts',(20.1661183969493,-20.5110918621599,-19.392441272119));
#79401=CARTESIAN_POINT('Ctrl Pts',(20.1753211256205,-20.502586809175,-19.3916925018503));
#79402=CARTESIAN_POINT('Ctrl Pts',(20.1797728982246,-20.4984367972524,-19.3913296634031));
#79403=CARTESIAN_POINT('Ctrl Pts',(20.1903914417592,-20.4884520946125,-19.3904626634993));
#79404=CARTESIAN_POINT('Ctrl Pts',(20.1965411645572,-20.4825993649006,-19.3899592823528));
#79405=CARTESIAN_POINT('Ctrl Pts',(20.2187191964895,-20.4612366821034,-19.3881391361993));
#79406=CARTESIAN_POINT('Ctrl Pts',(20.234537707751,-20.4455103275074,-19.3868317870986));
#79407=CARTESIAN_POINT('Ctrl Pts',(20.3782388263936,-20.2980581212227,-19.3748593846415));
#79408=CARTESIAN_POINT('Ctrl Pts',(20.4887239178553,-20.1504756742736,-19.365029261082));
#79409=CARTESIAN_POINT('Ctrl Pts',(20.6187517210273,-19.9194896954436,-19.3505852645999));
#79410=CARTESIAN_POINT('Ctrl Pts',(20.6545793194179,-19.8462585526793,-19.3461092757742));
#79411=CARTESIAN_POINT('Ctrl Pts',(20.7001745682777,-19.7376019264967,-19.3393714814267));
#79412=CARTESIAN_POINT('Ctrl Pts',(20.7133849161566,-19.703696624504,-19.337255711274));
#79413=CARTESIAN_POINT('Ctrl Pts',(20.7282518299472,-19.662425719248,-19.33464526405));
#79414=CARTESIAN_POINT('Ctrl Pts',(20.7307520027793,-19.6553679687156,-19.3341976301444));
#79415=CARTESIAN_POINT('Ctrl Pts',(20.7345842017419,-19.6443649257486,-19.3334976554587));
#79416=CARTESIAN_POINT('Ctrl Pts',(20.7359421452722,-19.6404286346189,-19.3332468233807));
#79417=CARTESIAN_POINT('Ctrl Pts',(20.7384412667097,-19.6331144696072,-19.3327799214073));
#79418=CARTESIAN_POINT('Ctrl Pts',(20.7395855275842,-19.6297377098414,-19.332564036783));
#79419=CARTESIAN_POINT('Ctrl Pts',(20.7421560610158,-19.6220884441896,-19.3320742636121));
#79420=CARTESIAN_POINT('Ctrl Pts',(20.7435772240377,-19.6178142895679,-19.3318000796951));
#79421=CARTESIAN_POINT('Ctrl Pts',(20.7478318299884,-19.6048808260464,-19.3309689225962));
#79422=CARTESIAN_POINT('Ctrl Pts',(20.7506229784018,-19.5962078613575,-19.3304095549054));
#79423=CARTESIAN_POINT('Ctrl Pts',(20.7716805003414,-19.5292975297536,-19.326080178729));
#79424=CARTESIAN_POINT('Ctrl Pts',(20.7874749007464,-19.4703180656595,-19.3221834057775));
#79425=CARTESIAN_POINT('Ctrl Pts',(20.8135917801933,-19.3526586091225,-19.3143577372729));
#79426=CARTESIAN_POINT('Ctrl Pts',(20.8240302306499,-19.2940562020501,-19.3104354811217));
#79427=CARTESIAN_POINT('Ctrl Pts',(20.8465428347647,-19.1272172980772,-19.2993134985049));
#79428=CARTESIAN_POINT('Ctrl Pts',(20.8527583288167,-19.0183698235923,-19.2921188905391));
#79429=CARTESIAN_POINT('Ctrl Pts',(20.8490716928712,-18.8346776074682,-19.2803153188366));
#79430=CARTESIAN_POINT('Ctrl Pts',(20.8436008343418,-18.759960260913,-19.2756059561699));
#79431=CARTESIAN_POINT('Ctrl Pts',(20.8318188580848,-18.667047596358,-19.2698686535368));
#79432=CARTESIAN_POINT('Ctrl Pts',(20.8292078886343,-18.6484447780359,-19.2687257837066));
#79433=CARTESIAN_POINT('Ctrl Pts',(20.8250486469854,-18.6214282864996,-19.2670740965107));
#79434=CARTESIAN_POINT('Ctrl Pts',(20.8236964948525,-18.6129857457606,-19.2665591017215));
#79435=CARTESIAN_POINT('Ctrl Pts',(20.8212348645011,-18.5981904410859,-19.2656585419943));
#79436=CARTESIAN_POINT('Ctrl Pts',(20.8201474438943,-18.5918341669058,-19.2652722826251));
#79437=CARTESIAN_POINT('Ctrl Pts',(20.8179785525398,-18.5794958455789,-19.2645237014159));
#79438=CARTESIAN_POINT('Ctrl Pts',(20.8169003266819,-18.5735132990433,-19.2641612806003));
#79439=CARTESIAN_POINT('Ctrl Pts',(20.8142595205016,-18.5592138782787,-19.2632962962392));
#79440=CARTESIAN_POINT('Ctrl Pts',(20.8126728040676,-18.5509015247552,-19.2627945047372));
#79441=CARTESIAN_POINT('Ctrl Pts',(20.8067569527533,-18.5208883293069,-19.2609862420577));
#79442=CARTESIAN_POINT('Ctrl Pts',(20.8021373881776,-18.49924570034,-19.2596890244646));
#79443=CARTESIAN_POINT('Ctrl Pts',(20.7556426527245,-18.2970051443598,-19.2476201150878));
#79444=CARTESIAN_POINT('Ctrl Pts',(20.6905574186346,-18.1225746712111,-19.237702832742));
#79445=CARTESIAN_POINT('Ctrl Pts',(20.5659197569792,-17.8879498976698,-19.2232203696414));
#79446=CARTESIAN_POINT('Ctrl Pts',(20.5242625130942,-17.8192640480971,-19.2188063243279));
#79447=CARTESIAN_POINT('Ctrl Pts',(20.4583862459383,-17.7233903089113,-19.2121526814936));
#79448=CARTESIAN_POINT('Ctrl Pts',(20.4372071578838,-17.6941944800549,-19.2100549595936));
#79449=CARTESIAN_POINT('Ctrl Pts',(20.4107559227381,-17.659624531298,-19.2074645333228));
#79450=CARTESIAN_POINT('Ctrl Pts',(20.4061863166082,-17.6537174054475,-19.2070180337968));
#79451=CARTESIAN_POINT('Ctrl Pts',(20.3990230156021,-17.6445579701804,-19.2063194511735));
#79452=CARTESIAN_POINT('Ctrl Pts',(20.3964507768393,-17.6412888503847,-19.2060688670949));
#79453=CARTESIAN_POINT('Ctrl Pts',(20.3916556988359,-17.6352314935894,-19.2056021863816));
#79454=CARTESIAN_POINT('Ctrl Pts',(20.3894354440697,-17.6324412838867,-19.2053862734997));
#79455=CARTESIAN_POINT('Ctrl Pts',(20.3843911162866,-17.6261348097701,-19.2048961250944));
#79456=CARTESIAN_POINT('Ctrl Pts',(20.3815628643992,-17.6226219701065,-19.2046215922564));
#79457=CARTESIAN_POINT('Ctrl Pts',(20.3742318633557,-17.6135758044634,-19.2039107753472));
#79458=CARTESIAN_POINT('Ctrl Pts',(20.3697123727214,-17.6080562053479,-19.2034733252998));
#79459=CARTESIAN_POINT('Ctrl Pts',(20.3417962865494,-17.574312033867,-19.2007764829244));
#79460=CARTESIAN_POINT('Ctrl Pts',(20.3176991783711,-17.5466781257956,-19.198470915906));
#79461=CARTESIAN_POINT('Ctrl Pts',(20.177474574603,-17.3940608236518,-19.185244408539));
#79462=CARTESIAN_POINT('Ctrl Pts',(20.0472904141954,-17.282849099074,-19.1737328150046));
#79463=CARTESIAN_POINT('Ctrl Pts',(19.8257629372119,-17.1357322821224,-19.1564516324388));
#79464=CARTESIAN_POINT('Ctrl Pts',(19.7428800537353,-17.0884174248192,-19.1503957283928));
#79465=CARTESIAN_POINT('Ctrl Pts',(19.6378354680984,-17.0375215562985,-19.1432258790296));
#79466=CARTESIAN_POINT('Ctrl Pts',(19.6184508683527,-17.02848941284,-19.1419224643709));
#79467=CARTESIAN_POINT('Ctrl Pts',(19.5907098734763,-17.0160717096726,-19.1400843555826));
#79468=CARTESIAN_POINT('Ctrl Pts',(19.582464069937,-17.0124436387284,-19.1395413598245));
#79469=CARTESIAN_POINT('Ctrl Pts',(19.5682051399277,-17.0062781867502,-19.1386081095363));
#79470=CARTESIAN_POINT('Ctrl Pts',(19.5622030256673,-17.0037157959389,-19.1382170045572));
#79471=CARTESIAN_POINT('Ctrl Pts',(19.5506923729632,-16.9988645339206,-19.1374702340522));
#79472=CARTESIAN_POINT('Ctrl Pts',(19.5451858307565,-16.9965711135368,-19.1371144167087));
#79473=CARTESIAN_POINT('Ctrl Pts',(19.530851145094,-16.9906718303984,-19.1361918113652));
#79474=CARTESIAN_POINT('Ctrl Pts',(19.52200813731,-16.9871022631275,-19.1356262555011));
#79475=CARTESIAN_POINT('Ctrl Pts',(19.4918208589233,-16.9751534402262,-19.1337075830069));
#79476=CARTESIAN_POINT('Ctrl Pts',(19.4703642364132,-16.9670610722524,-19.1323640975923));
#79477=CARTESIAN_POINT('Ctrl Pts',(19.2828331497991,-16.8997932065347,-19.1207863983065));
#79478=CARTESIAN_POINT('Ctrl Pts',(19.1101036752726,-16.8612290332538,-19.1113112693238));
#79479=CARTESIAN_POINT('Ctrl Pts',(18.8485362089927,-16.8363344380779,-19.0970129366175));
#79480=CARTESIAN_POINT('Ctrl Pts',(18.7620798226963,-16.8334230071062,-19.0922794870084));
#79481=CARTESIAN_POINT('Ctrl Pts',(18.6380318912868,-16.8368407315622,-19.085193286206));
#79482=CARTESIAN_POINT('Ctrl Pts',(18.6004054886259,-16.83888364723,-19.0830044536186));
#79483=CARTESIAN_POINT('Ctrl Pts',(18.5553177162121,-16.8425406270373,-19.0803129940251));
#79484=CARTESIAN_POINT('Ctrl Pts',(18.5477825515759,-16.8431924547958,-19.079860883827));
#79485=CARTESIAN_POINT('Ctrl Pts',(18.5360882550953,-16.8442672329068,-19.0791554174678));
#79486=CARTESIAN_POINT('Ctrl Pts',(18.531926522962,-16.844662156788,-19.0789036084861));
#79487=CARTESIAN_POINT('Ctrl Pts',(18.5242190415939,-16.8454165928799,-19.0784358269419));
#79488=CARTESIAN_POINT('Ctrl Pts',(18.5206730202344,-16.8457727328742,-19.078220045606));
#79489=CARTESIAN_POINT('Ctrl Pts',(18.5126690300257,-16.8465970233165,-19.0777317141393));
#79490=CARTESIAN_POINT('Ctrl Pts',(18.5082116643118,-16.8470703766849,-19.0774588761457));
#79491=CARTESIAN_POINT('Ctrl Pts',(18.4950909112337,-16.8485059002243,-19.0766531940646));
#79492=CARTESIAN_POINT('Ctrl Pts',(18.4864320471011,-16.8495074118605,-19.0761182152734));
#79493=CARTESIAN_POINT('Ctrl Pts',(18.4248767052849,-16.857012617993,-19.072292922822));
#79494=CARTESIAN_POINT('Ctrl Pts',(18.3722406731706,-16.8654577650984,-19.0689057252391));
#79495=CARTESIAN_POINT('Ctrl Pts',(18.3023589698188,-16.8793934208461,-19.0643005646603));
#79496=CARTESIAN_POINT('Ctrl Pts',(18.2847793266029,-16.8831324905262,-19.0631327684647));
#79497=CARTESIAN_POINT('Ctrl Pts',(18.2202253666096,-16.8977242381343,-19.0588147274084));
#79498=CARTESIAN_POINT('Ctrl Pts',(18.1735789140705,-16.9099565985596,-19.0556364797295));
#79499=CARTESIAN_POINT('Ctrl Pts',(18.0225990610318,-16.9551120277866,-19.0452266588094));
#79500=CARTESIAN_POINT('Ctrl Pts',(17.9203845395124,-16.9945306597934,-19.0379941005091));
#79501=CARTESIAN_POINT('Ctrl Pts',(17.7533799965462,-17.0742885084566,-19.0260981496392));
#79502=CARTESIAN_POINT('Ctrl Pts',(17.6868830803873,-17.1105428615085,-19.0213353689672));
#79503=CARTESIAN_POINT('Ctrl Pts',(17.6063835861017,-17.1602055849986,-19.0155404373673));
#79504=CARTESIAN_POINT('Ctrl Pts',(17.5904361796315,-17.1703412707252,-19.0143907435225));
#79505=CARTESIAN_POINT('Ctrl Pts',(17.5674553626784,-17.1853828770944,-19.0127310753828));
#79506=CARTESIAN_POINT('Ctrl Pts',(17.5603130230162,-17.1901199435717,-19.0122148394162));
#79507=CARTESIAN_POINT('Ctrl Pts',(17.547844701473,-17.1984988645741,-19.011312847506));
#79508=CARTESIAN_POINT('Ctrl Pts',(17.5425062721063,-17.2021219122513,-19.0109263903223));
#79509=CARTESIAN_POINT('Ctrl Pts',(17.5321751546603,-17.2092025587906,-19.0101779606139));
#79510=CARTESIAN_POINT('Ctrl Pts',(17.527180623417,-17.2126573444407,-19.0098158865991));
#79511=CARTESIAN_POINT('Ctrl Pts',(17.5152807732225,-17.2209645659733,-19.008952579822));
#79512=CARTESIAN_POINT('Ctrl Pts',(17.5083894353648,-17.2258369212145,-19.0084521122372));
#79513=CARTESIAN_POINT('Ctrl Pts',(17.4836527617036,-17.2435492124087,-19.0066536141676));
#79514=CARTESIAN_POINT('Ctrl Pts',(17.4659781640409,-17.2566260038337,-19.005364705296));
#79515=CARTESIAN_POINT('Ctrl Pts',(17.3000937233961,-17.383403510882,-18.9932203621058));
#79516=CARTESIAN_POINT('Ctrl Pts',(17.167345780027,-17.5159698428672,-18.983234834381));
#79517=CARTESIAN_POINT('Ctrl Pts',(17.00544248396,-17.7272249387109,-18.9687214708651));
#79518=CARTESIAN_POINT('Ctrl Pts',(16.9607585718426,-17.7928632905634,-18.9643555302891));
#79519=CARTESIAN_POINT('Ctrl Pts',(16.9014073609634,-17.89153974784,-18.9577673284734));
#79520=CARTESIAN_POINT('Ctrl Pts',(16.8837304163383,-17.9226925376627,-18.9556837510472));
#79521=CARTESIAN_POINT('Ctrl Pts',(16.8633406756185,-17.9608500406276,-18.9531090179757));
#79522=CARTESIAN_POINT('Ctrl Pts',(16.8598628566578,-17.9674419701935,-18.9526634156439));
#79523=CARTESIAN_POINT('Ctrl Pts',(16.8544998953419,-17.9777384166141,-18.9519659341345));
#79524=CARTESIAN_POINT('Ctrl Pts',(16.8525906926019,-17.9814304282409,-18.9517155463365));
#79525=CARTESIAN_POINT('Ctrl Pts',(16.849063646917,-17.9883005330516,-18.9512490401501));
#79526=CARTESIAN_POINT('Ctrl Pts',(16.8474429570878,-17.9914771002208,-18.9510331043112));
#79527=CARTESIAN_POINT('Ctrl Pts',(16.8437888034243,-17.9986842011171,-18.9505426562364));
#79528=CARTESIAN_POINT('Ctrl Pts',(16.8417602112045,-18.0027171333653,-18.9502678451362));
#79529=CARTESIAN_POINT('Ctrl Pts',(16.8357860256382,-18.0146893217936,-18.9494510214997));
#79530=CARTESIAN_POINT('Ctrl Pts',(16.8318774456107,-18.0226467938838,-18.9489067869505));
#79531=CARTESIAN_POINT('Ctrl Pts',(16.80314318914,-18.0820874656696,-18.9448329603227));
#79532=CARTESIAN_POINT('Ctrl Pts',(16.7803638034158,-18.1345281594861,-18.9411920259084));
#79533=CARTESIAN_POINT('Ctrl Pts',(16.6996314218625,-18.3431009769142,-18.926702986597));
#79534=CARTESIAN_POINT('Ctrl Pts',(16.6580537910332,-18.5049334714458,-18.915500136708));
#79535=CARTESIAN_POINT('Ctrl Pts',(16.6280919357943,-18.7278383788809,-18.9010061658868));
#79536=CARTESIAN_POINT('Ctrl Pts',(16.6227108984473,-18.7859984880139,-18.8973011289853));
#79537=CARTESIAN_POINT('Ctrl Pts',(16.6179213248027,-18.8800322479673,-18.8914414370162));
#79538=CARTESIAN_POINT('Ctrl Pts',(16.6170073710083,-18.9157954316116,-18.8892429293612));
#79539=CARTESIAN_POINT('Ctrl Pts',(16.616997796834,-18.9625398028534,-18.8864068425017));
#79540=CARTESIAN_POINT('Ctrl Pts',(16.6170808697117,-18.9735132186089,-18.8857437458361));
#79541=CARTESIAN_POINT('Ctrl Pts',(16.6173556708795,-18.9914191387053,-18.8846659965562));
#79542=CARTESIAN_POINT('Ctrl Pts',(16.6174961452131,-18.9983521191167,-18.8842497461034));
#79543=CARTESIAN_POINT('Ctrl Pts',(16.6178328488767,-19.0117251986035,-18.8834488062694));
#79544=CARTESIAN_POINT('Ctrl Pts',(16.6180244184857,-19.0181653284832,-18.8830639754413));
#79545=CARTESIAN_POINT('Ctrl Pts',(16.6185373485208,-19.0331125219242,-18.882172803864));
#79546=CARTESIAN_POINT('Ctrl Pts',(16.6188806293231,-19.0416187593832,-18.8816671552148));
#79547=CARTESIAN_POINT('Ctrl Pts',(16.620136566466,-19.0686864914159,-18.8800627579892));
#79548=CARTESIAN_POINT('Ctrl Pts',(16.6212423368452,-19.0872384645813,-18.8789700600468));
#79549=CARTESIAN_POINT('Ctrl Pts',(16.6243860729691,-19.1304038377679,-18.8764423790067));
#79550=CARTESIAN_POINT('Ctrl Pts',(16.6266107498987,-19.155001158676,-18.8750131988553));
#79551=CARTESIAN_POINT('Ctrl Pts',(16.6359173603785,-19.2410813321558,-18.8700446047059));
#79552=CARTESIAN_POINT('Ctrl Pts',(16.6452642973998,-19.3022896030012,-18.8665717716127));
#79553=CARTESIAN_POINT('Ctrl Pts',(16.6784970300946,-19.4702077849289,-18.8571027638153));
#79554=CARTESIAN_POINT('Ctrl Pts',(16.7079721266401,-19.5755543888119,-18.8512347660574));
#79555=CARTESIAN_POINT('Ctrl Pts',(16.7454194032426,-19.6781103292199,-18.8452753983371));
#79556=CARTESIAN_POINT('Origin',(18.734,-18.952,0.));
#79557=CARTESIAN_POINT('',(16.7454193872878,-19.6781102855251,-18.0457833417799));
#79558=CARTESIAN_POINT('',(16.745419450845,-19.6781104595875,-18.2676549380821));
#79559=CARTESIAN_POINT('',(16.7454194499637,-19.6781104571739,0.));
#79560=CARTESIAN_POINT('',(16.6170000023184,-18.9519009238278,-18.3109437209775));
#79561=CARTESIAN_POINT('Ctrl Pts',(16.745419450845,-19.6781104595875,-18.2676549380821));
#79562=CARTESIAN_POINT('Ctrl Pts',(16.7423111909751,-19.6695979460473,-18.2681610694787));
#79563=CARTESIAN_POINT('Ctrl Pts',(16.7392574281066,-19.6610650299046,-18.2686659571902));
#79564=CARTESIAN_POINT('Ctrl Pts',(16.7027368374843,-19.5569145222169,-18.2748002898151));
#79565=CARTESIAN_POINT('Ctrl Pts',(16.6761195712795,-19.4590312384636,-18.2802690475673));
#79566=CARTESIAN_POINT('Ctrl Pts',(16.6333078555506,-19.240845234103,-18.2923592474485));
#79567=CARTESIAN_POINT('Ctrl Pts',(16.6202348295939,-19.1203084927762,-18.2989763297896));
#79568=CARTESIAN_POINT('Ctrl Pts',(16.6172719191199,-18.987828630187,-18.3067856556148));
#79569=CARTESIAN_POINT('Ctrl Pts',(16.6171084239076,-18.9763207955218,-18.3074684926059));
#79570=CARTESIAN_POINT('Ctrl Pts',(16.6170172119703,-18.9612501741062,-18.3083692643783));
#79571=CARTESIAN_POINT('Ctrl Pts',(16.6170046437052,-18.9576878419957,-18.3085826629695));
#79572=CARTESIAN_POINT('Ctrl Pts',(16.6170002821642,-18.953343794759,-18.3088434905605));
#79573=CARTESIAN_POINT('Ctrl Pts',(16.6169999302839,-18.9525620664735,-18.3088904512387));
#79574=CARTESIAN_POINT('Ctrl Pts',(16.617000011396,-18.9517803397697,-18.3089374357138));
#79575=CARTESIAN_POINT('Ctrl Pts',(16.6170000023184,-18.9519009238278,-18.3109437209775));
#79576=CARTESIAN_POINT('Ctrl Pts',(16.6170002492315,-18.9466250329454,-18.3112630160645));
#79577=CARTESIAN_POINT('Ctrl Pts',(16.6170202186042,-18.9413491960951,-18.3115823111514));
#79578=CARTESIAN_POINT('Ctrl Pts',(16.6170599094811,-18.936073507803,-18.3119016062384));
#79579=CARTESIAN_POINT('Ctrl Pts',(16.6176053981758,-18.8635674674004,-18.3162898151688));
#79580=CARTESIAN_POINT('Ctrl Pts',(16.6218813020779,-18.7909479534649,-18.3206780240991));
#79581=CARTESIAN_POINT('Ctrl Pts',(16.6299021760198,-18.7186304494543,-18.3250662330295));
#79582=CARTESIAN_POINT('Ctrl Pts',(16.6379111456549,-18.6464202766101,-18.3294479291303));
#79583=CARTESIAN_POINT('Ctrl Pts',(16.6496539988946,-18.5745116993623,-18.333829625231));
#79584=CARTESIAN_POINT('Ctrl Pts',(16.6650932824123,-18.5033197197107,-18.3382113213318));
#79585=CARTESIAN_POINT('Ctrl Pts',(16.6805144235431,-18.4322113963008,-18.3425878685909));
#79586=CARTESIAN_POINT('Ctrl Pts',(16.6996232646345,-18.3618184668105,-18.34696441585));
#79587=CARTESIAN_POINT('Ctrl Pts',(16.7223308201355,-18.2925486289473,-18.3513409631092));
#79588=CARTESIAN_POINT('Ctrl Pts',(16.7450239748349,-18.2233227210085,-18.3557147348256));
#79589=CARTESIAN_POINT('Ctrl Pts',(16.7713111657669,-18.155218948753,-18.3600885065421));
#79590=CARTESIAN_POINT('Ctrl Pts',(16.8010531665404,-18.0886312844337,-18.3644622782586));
#79591=CARTESIAN_POINT('Ctrl Pts',(16.8307861167232,-18.0220638829642,-18.3688347190216));
#79592=CARTESIAN_POINT('Ctrl Pts',(16.8639715929645,-17.9570121136705,-18.3732071597847));
#79593=CARTESIAN_POINT('Ctrl Pts',(16.9004223233176,-17.8938497726825,-18.3775796005477));
#79594=CARTESIAN_POINT('Ctrl Pts',(16.93687398572,-17.8306858166264,-18.3819521531146));
#79595=CARTESIAN_POINT('Ctrl Pts',(16.9765908251607,-17.7694118015945,-18.3863247056814));
#79596=CARTESIAN_POINT('Ctrl Pts',(17.0193405651388,-17.7103752489413,-18.3906972582483));
#79597=CARTESIAN_POINT('Ctrl Pts',(17.0621346724097,-17.6512774259268,-18.3950743488151));
#79598=CARTESIAN_POINT('Ctrl Pts',(17.1079676812098,-17.5944220931023,-18.3994514393819));
#79599=CARTESIAN_POINT('Ctrl Pts',(17.1565655683569,-17.5401254964174,-18.4038285299488));
#79600=CARTESIAN_POINT('Ctrl Pts',(17.2051899966138,-17.4857992463457,-18.4082080110073));
#79601=CARTESIAN_POINT('Ctrl Pts',(17.2565819695237,-17.4340348572235,-18.4125874920657));
#79602=CARTESIAN_POINT('Ctrl Pts',(17.3104308762818,-17.3851113791988,-18.4169669731242));
#79603=CARTESIAN_POINT('Ctrl Pts',(17.3643752298659,-17.3361011846376,-18.4213542167834));
#79604=CARTESIAN_POINT('Ctrl Pts',(17.4207848402037,-17.2899422626056,-18.4257414604427));
#79605=CARTESIAN_POINT('Ctrl Pts',(17.4793168103112,-17.2468727046017,-18.4301287041019));
#79606=CARTESIAN_POINT('Ctrl Pts',(17.5191129099215,-17.2175895552844,-18.4331116070413));
#79607=CARTESIAN_POINT('Ctrl Pts',(17.5598894741973,-17.1897336331319,-18.4360945099806));
#79608=CARTESIAN_POINT('Ctrl Pts',(17.6015321394767,-17.1633676887404,-18.4390774129199));
#79609=CARTESIAN_POINT('Ctrl Pts',(17.6627935078073,-17.1245802139255,-18.4434656218502));
#79610=CARTESIAN_POINT('Ctrl Pts',(17.7261694924203,-17.0888680068776,-18.4478538307805));
#79611=CARTESIAN_POINT('Ctrl Pts',(17.7913186157342,-17.0564681992225,-18.4522420397107));
#79612=CARTESIAN_POINT('Ctrl Pts',(17.8563710469469,-17.0241164782541,-18.4566237358114));
#79613=CARTESIAN_POINT('Ctrl Pts',(17.9231909643683,-16.995067610473,-18.461005431912));
#79614=CARTESIAN_POINT('Ctrl Pts',(17.9914091442163,-16.96951473627,-18.4653871280127));
#79615=CARTESIAN_POINT('Ctrl Pts',(18.0595471622739,-16.9439918887279,-18.4697636752717));
#79616=CARTESIAN_POINT('Ctrl Pts',(18.1290797293045,-16.9219570424211,-18.4741402225307));
#79617=CARTESIAN_POINT('Ctrl Pts',(18.1996158698649,-16.9035560536203,-18.4785167697897));
#79618=CARTESIAN_POINT('Ctrl Pts',(18.27010727743,-16.8851667344591,-18.482890541506));
#79619=CARTESIAN_POINT('Ctrl Pts',(18.3416005301139,-16.8704068217632,-18.4872643132223));
#79620=CARTESIAN_POINT('Ctrl Pts',(18.4136889989943,-16.8593724978786,-18.4916380849387));
#79621=CARTESIAN_POINT('Ctrl Pts',(18.4857555311115,-16.8483415317759,-18.4960105257016));
#79622=CARTESIAN_POINT('Ctrl Pts',(18.5584164432962,-16.8410339766644,-18.5003829664645));
#79623=CARTESIAN_POINT('Ctrl Pts',(18.6312560654047,-16.8374946952292,-18.5047554072274));
#79624=CARTESIAN_POINT('Ctrl Pts',(18.7040975500304,-16.8339553232942,-18.5091279597941));
#79625=CARTESIAN_POINT('Ctrl Pts',(18.7771172717463,-16.8341844377533,-18.5135005123608));
#79626=CARTESIAN_POINT('Ctrl Pts',(18.8498972932256,-16.8381748375462,-18.5178730649275));
#79627=CARTESIAN_POINT('Ctrl Pts',(18.9227528485563,-16.8421693787264,-18.5222501554942));
#79628=CARTESIAN_POINT('Ctrl Pts',(18.9953677242796,-16.8499329725836,-18.5266272460608));
#79629=CARTESIAN_POINT('Ctrl Pts',(19.0673276840478,-16.8614063869209,-18.5310043366275));
#79630=CARTESIAN_POINT('Ctrl Pts',(19.1393269438208,-16.8728860673155,-18.5353838176858));
#79631=CARTESIAN_POINT('Ctrl Pts',(19.2106701033887,-16.8880795015321,-18.5397632987441));
#79632=CARTESIAN_POINT('Ctrl Pts',(19.2809543980004,-16.9068765595916,-18.5441427798024));
#79633=CARTESIAN_POINT('Ctrl Pts',(19.3513632710527,-16.9257069353104,-18.5485300234615));
#79634=CARTESIAN_POINT('Ctrl Pts',(19.4207090718553,-16.9481535415649,-18.5529172671205));
#79635=CARTESIAN_POINT('Ctrl Pts',(19.4886059995026,-16.974056930669,-18.5573045107796));
#79636=CARTESIAN_POINT('Ctrl Pts',(19.5347693678658,-16.9916687392515,-18.5602874137202));
#79637=CARTESIAN_POINT('Ctrl Pts',(19.580263370974,-17.010877494452,-18.5632703166607));
#79638=CARTESIAN_POINT('Ctrl Pts',(19.6249733426251,-17.0316210002368,-18.5662532196012));
#79639=CARTESIAN_POINT('Ctrl Pts',(19.6907470875151,-17.0621371917536,-18.5706414285353));
#79640=CARTESIAN_POINT('Ctrl Pts',(19.7550796205675,-17.0960960250392,-18.5750296374695));
#79641=CARTESIAN_POINT('Ctrl Pts',(19.817586716273,-17.1333387263383,-18.5794178464036));
#79642=CARTESIAN_POINT('Ctrl Pts',(19.8800010410849,-17.1705261532939,-18.5837995425081));
#79643=CARTESIAN_POINT('Ctrl Pts',(19.9405948958111,-17.2109875282316,-18.5881812386125));
#79644=CARTESIAN_POINT('Ctrl Pts',(19.9990060261177,-17.2545169356115,-18.592562934717));
#79645=CARTESIAN_POINT('Ctrl Pts',(20.0573485186977,-17.2979951924735,-18.5969394819799));
#79646=CARTESIAN_POINT('Ctrl Pts',(20.1135129971313,-17.3445340332472,-18.6013160292427));
#79647=CARTESIAN_POINT('Ctrl Pts',(20.1671651917851,-17.3938836586905,-18.6056925765056));
#79648=CARTESIAN_POINT('Ctrl Pts',(20.2207833609968,-17.4432019873186,-18.6100663482258));
#79649=CARTESIAN_POINT('Ctrl Pts',(20.2718920534934,-17.495327238032,-18.614440119946));
#79650=CARTESIAN_POINT('Ctrl Pts',(20.3201902946194,-17.549969561937,-18.6188138916661));
#79651=CARTESIAN_POINT('Ctrl Pts',(20.3684738384283,-17.6045952579991,-18.6231863324329));
#79652=CARTESIAN_POINT('Ctrl Pts',(20.413948309488,-17.6617361453877,-18.6275587731997));
#79653=CARTESIAN_POINT('Ctrl Pts',(20.4563509910147,-17.7210669946131,-18.6319312139664));
#79654=CARTESIAN_POINT('Ctrl Pts',(20.4987547567825,-17.7803993609347,-18.6363037665369));
#79655=CARTESIAN_POINT('Ctrl Pts',(20.5380862982194,-17.8419214066551,-18.6406763191075));
#79656=CARTESIAN_POINT('Ctrl Pts',(20.5741254487293,-17.9052778148243,-18.645048871678));
#79657=CARTESIAN_POINT('Ctrl Pts',(20.6102020020285,-17.968699976663,-18.6494259622485));
#79658=CARTESIAN_POINT('Ctrl Pts',(20.6429791031795,-18.0339598817704,-18.653803052819));
#79659=CARTESIAN_POINT('Ctrl Pts',(20.6722823388073,-18.1006771616669,-18.6581801433894));
#79660=CARTESIAN_POINT('Ctrl Pts',(20.7016015780196,-18.1674308783458,-18.6625596244515));
#79661=CARTESIAN_POINT('Ctrl Pts',(20.7274430033788,-18.2356431030904,-18.6669391055136));
#79662=CARTESIAN_POINT('Ctrl Pts',(20.7496812078476,-18.3049155632146,-18.6713185865757));
#79663=CARTESIAN_POINT('Ctrl Pts',(20.7719588293843,-18.3743108083083,-18.6757058302384));
#79664=CARTESIAN_POINT('Ctrl Pts',(20.7906203524691,-18.4447695748772,-18.6800930739012));
#79665=CARTESIAN_POINT('Ctrl Pts',(20.8055910206598,-18.5158811594051,-18.684480317564));
#79666=CARTESIAN_POINT('Ctrl Pts',(20.8157696323546,-18.564230184091,-18.6874632204702));
#79667=CARTESIAN_POINT('Ctrl Pts',(20.8242431499881,-18.6128807754351,-18.6904461233765));
#79668=CARTESIAN_POINT('Ctrl Pts',(20.8310018039417,-18.6617028517791,-18.6934290262827));
#79669=CARTESIAN_POINT('Ctrl Pts',(20.8409445967655,-18.7335259978741,-18.6978172352092));
#79670=CARTESIAN_POINT('Ctrl Pts',(20.8472125720512,-18.8060007495856,-18.7022054441356));
#79671=CARTESIAN_POINT('Ctrl Pts',(20.8497312594192,-18.8787180928442,-18.7065936530621));
#79672=CARTESIAN_POINT('Ctrl Pts',(20.8522462086376,-18.9513275115089,-18.7109753491589));
#79673=CARTESIAN_POINT('Ctrl Pts',(20.8510228997993,-19.0241783288765,-18.7153570452558));
#79674=CARTESIAN_POINT('Ctrl Pts',(20.8460383938856,-19.096854488205,-18.7197387413526));
#79675=CARTESIAN_POINT('Ctrl Pts',(20.841059745163,-19.1694452472631,-18.7241152886079));
#79676=CARTESIAN_POINT('Ctrl Pts',(20.8323287119819,-19.2418612771284,-18.7284918358631));
#79677=CARTESIAN_POINT('Ctrl Pts',(20.8198744021603,-19.3136862983475,-18.7328683831184));
#79678=CARTESIAN_POINT('Ctrl Pts',(20.8074279906809,-19.3854657691824,-18.737242154831));
#79679=CARTESIAN_POINT('Ctrl Pts',(20.7912630697939,-19.4566545009247,-18.7416159265437));
#79680=CARTESIAN_POINT('Ctrl Pts',(20.7714604446763,-19.5268425318116,-18.7459896982563));
#79681=CARTESIAN_POINT('Ctrl Pts',(20.7516638455638,-19.5970092042456,-18.7503621390155));
#79682=CARTESIAN_POINT('Ctrl Pts',(20.728231870793,-19.6661753164087,-18.7547345797747));
#79683=CARTESIAN_POINT('Ctrl Pts',(20.7012957832833,-19.7339439245084,-18.759107020534));
#79684=CARTESIAN_POINT('Ctrl Pts',(20.6743590070147,-19.8017142654596,-18.763479573097));
#79685=CARTESIAN_POINT('Ctrl Pts',(20.6439181201448,-19.8680865838727,-18.7678521256601));
#79686=CARTESIAN_POINT('Ctrl Pts',(20.6101527159953,-19.9326834281578,-18.7722246782232));
#79687=CARTESIAN_POINT('Ctrl Pts',(20.5763522688351,-19.9973473134859,-18.7766017687863));
#79688=CARTESIAN_POINT('Ctrl Pts',(20.5392206395556,-20.0602316172898,-18.7809788593495));
#79689=CARTESIAN_POINT('Ctrl Pts',(20.4989832512011,-20.1209837992802,-18.7853559499126));
#79690=CARTESIAN_POINT('Ctrl Pts',(20.458723887715,-20.1817691602927,-18.7897354309674));
#79691=CARTESIAN_POINT('Ctrl Pts',(20.4153556750915,-20.2404196929921,-18.7941149120222));
#79692=CARTESIAN_POINT('Ctrl Pts',(20.3691456171804,-20.2966143724562,-18.798494393077));
#79693=CARTESIAN_POINT('Ctrl Pts',(20.3228536522506,-20.352908656614,-18.8028816367327));
#79694=CARTESIAN_POINT('Ctrl Pts',(20.2737101085666,-20.4067380382461,-18.8072688803884));
#79695=CARTESIAN_POINT('Ctrl Pts',(20.2220198585457,-20.4578173529926,-18.8116561240441));
#79696=CARTESIAN_POINT('Ctrl Pts',(20.1868754689055,-20.4925463655101,-18.8146390270174));
#79697=CARTESIAN_POINT('Ctrl Pts',(20.1505545743005,-20.5260048960148,-18.8176219299908));
#79698=CARTESIAN_POINT('Ctrl Pts',(20.1131612647177,-20.5581143190639,-18.8206048329642));
#79699=CARTESIAN_POINT('Ctrl Pts',(20.0581512102737,-20.6053511411,-18.8249930418924));
#79700=CARTESIAN_POINT('Ctrl Pts',(20.0006041495887,-20.6498507249,-18.8293812508206));
#79701=CARTESIAN_POINT('Ctrl Pts',(19.9408236893631,-20.6913290611014,-18.8337694597489));
#79702=CARTESIAN_POINT('Ctrl Pts',(19.8811319532531,-20.7327458365742,-18.8381511558474));
#79703=CARTESIAN_POINT('Ctrl Pts',(19.8192137908502,-20.7711499931519,-18.8425328519459));
#79704=CARTESIAN_POINT('Ctrl Pts',(19.7554066235765,-20.8062970391267,-18.8469145480445));
#79705=CARTESIAN_POINT('Ctrl Pts',(19.6916744348034,-20.8414027845247,-18.8512910953013));
#79706=CARTESIAN_POINT('Ctrl Pts',(19.626058071091,-20.8732587908218,-18.8556676425582));
#79707=CARTESIAN_POINT('Ctrl Pts',(19.5589233130916,-20.9016642089134,-18.860044189815));
#79708=CARTESIAN_POINT('Ctrl Pts',(19.4918311309808,-20.9300516127014,-18.8644179615291));
#79709=CARTESIAN_POINT('Ctrl Pts',(19.4232229083438,-20.9549925826767,-18.8687917332433));
#79710=CARTESIAN_POINT('Ctrl Pts',(19.3534870964552,-20.9763331586786,-18.8731655049574));
#79711=CARTESIAN_POINT('Ctrl Pts',(19.2837725054089,-20.9976672406713,-18.8775379457181));
#79712=CARTESIAN_POINT('Ctrl Pts',(19.2129314673137,-21.0154029627471,-18.8819103864787));
#79713=CARTESIAN_POINT('Ctrl Pts',(19.1413687992101,-21.0294358381019,-18.8862828272394));
#79714=CARTESIAN_POINT('Ctrl Pts',(19.0698043012416,-21.0434690722788,-18.8906553798038));
#79715=CARTESIAN_POINT('Ctrl Pts',(18.9975186103771,-21.0537991808917,-18.8950279323683));
#79716=CARTESIAN_POINT('Ctrl Pts',(18.9249263141295,-21.0603728661157,-18.8994004849327));
#79717=CARTESIAN_POINT('Ctrl Pts',(18.8522586788592,-21.0669533737582,-18.9037775754971));
#79718=CARTESIAN_POINT('Ctrl Pts',(18.7792842843246,-21.0697696306809,-18.9081546660614));
#79719=CARTESIAN_POINT('Ctrl Pts',(18.706421578337,-21.0688203586177,-18.9125317566258));
#79720=CARTESIAN_POINT('Ctrl Pts',(18.6335190793216,-21.0678705681219,-18.9169112376818));
#79721=CARTESIAN_POINT('Ctrl Pts',(18.5607288719989,-21.0631511854097,-18.9212907187378));
#79722=CARTESIAN_POINT('Ctrl Pts',(18.4884654116451,-21.0547129537627,-18.9256701997938));
#79723=CARTESIAN_POINT('Ctrl Pts',(18.4160738647929,-21.0462597654067,-18.9300574434505));
#79724=CARTESIAN_POINT('Ctrl Pts',(18.3442114053898,-21.0340746456018,-18.9344446871072));
#79725=CARTESIAN_POINT('Ctrl Pts',(18.2732828331918,-21.0182595897438,-18.938831930764));
#79726=CARTESIAN_POINT('Ctrl Pts',(18.22505823831,-21.0075068755956,-18.9418148337245));
#79727=CARTESIAN_POINT('Ctrl Pts',(18.1772650979154,-20.9950772191552,-18.944797736685));
#79728=CARTESIAN_POINT('Ctrl Pts',(18.1300258654971,-20.9810155851672,-18.9477806396456));
#79729=CARTESIAN_POINT('Ctrl Pts',(18.0605280442509,-20.9603282692373,-18.9521690525416));
#79730=CARTESIAN_POINT('Ctrl Pts',(17.9919586602188,-20.9360257809644,-18.9565574654377));
#79731=CARTESIAN_POINT('Ctrl Pts',(17.9247209128513,-20.9082096920074,-18.9609458783338));
#79732=CARTESIAN_POINT('Ctrl Pts',(17.8574469480808,-20.8803786200008,-18.9653366550348));
#79733=CARTESIAN_POINT('Ctrl Pts',(17.7915065313157,-20.8490302580147,-18.9697274317358));
#79734=CARTESIAN_POINT('Ctrl Pts',(17.7272902809765,-20.8143169820478,-18.9741182084367));
#79735=CARTESIAN_POINT('Ctrl Pts',(17.6632831695812,-20.779716759986,-18.9784946852931));
#79736=CARTESIAN_POINT('Ctrl Pts',(17.6009894538961,-20.7417737029155,-18.9828711621495));
#79737=CARTESIAN_POINT('Ctrl Pts',(17.5407759393722,-20.7006867475734,-18.9872476390058));
#79738=CARTESIAN_POINT('Ctrl Pts',(17.4806016974324,-20.659626590051,-18.9916212614273));
#79739=CARTESIAN_POINT('Ctrl Pts',(17.4225053614458,-20.6154268749417,-18.9959948838488));
#79740=CARTESIAN_POINT('Ctrl Pts',(17.3668265523033,-20.5683309574197,-19.0003685062703));
#79741=CARTESIAN_POINT('Ctrl Pts',(17.3111656906036,-20.521250220741,-19.0047407189034));
#79742=CARTESIAN_POINT('Ctrl Pts',(17.2579211759187,-20.4712754472109,-19.0091129315366));
#79743=CARTESIAN_POINT('Ctrl Pts',(17.207399864766,-20.4186905014704,-19.0134851441697));
#79744=CARTESIAN_POINT('Ctrl Pts',(17.1565195529559,-20.3657318910396,-19.0178884254187));
#79745=CARTESIAN_POINT('Ctrl Pts',(17.1084016691149,-20.3101261971702,-19.0222917066677));
#79746=CARTESIAN_POINT('Ctrl Pts',(17.0633209237031,-20.2522001476787,-19.0266949879167));
#79747=CARTESIAN_POINT('Ctrl Pts',(17.0185206470214,-20.1946344836554,-19.0310708742615));
#79748=CARTESIAN_POINT('Ctrl Pts',(16.9767200691604,-20.134777679211,-19.0354467606063));
#79749=CARTESIAN_POINT('Ctrl Pts',(16.9381461790676,-20.0729808445475,-19.0398226469511));
#79750=CARTESIAN_POINT('Ctrl Pts',(16.8992100556101,-20.0106036982979,-19.0442396256522));
#79751=CARTESIAN_POINT('Ctrl Pts',(16.8635617987445,-19.9462503235747,-19.0486566043533));
#79752=CARTESIAN_POINT('Ctrl Pts',(16.8313871436981,-19.8803066944898,-19.0530735830544));
#79753=CARTESIAN_POINT('Ctrl Pts',(16.7992124886517,-19.814363065405,-19.0574905617554));
#79754=CARTESIAN_POINT('Ctrl Pts',(16.7705115857647,-19.7468296619722,-19.0619075404565));
#79755=CARTESIAN_POINT('Ctrl Pts',(16.7454194499637,-19.6781104571739,-19.0663245191576));
#79756=CARTESIAN_POINT('',(16.617000908626,-18.9539458502908,-18.0890147563015));
#79757=CARTESIAN_POINT('Ctrl Pts',(16.7454194032426,-19.6781103292199,-18.8452753983371));
#79758=CARTESIAN_POINT('Ctrl Pts',(16.7566881939313,-19.7089718906256,-18.8434820805428));
#79759=CARTESIAN_POINT('Ctrl Pts',(16.7686789069382,-19.7395806962145,-18.8416796834934));
#79760=CARTESIAN_POINT('Ctrl Pts',(16.8104694161502,-19.8393480406311,-18.8356907683221));
#79761=CARTESIAN_POINT('Ctrl Pts',(16.8432351201276,-19.9071764613245,-18.8314361897634));
#79762=CARTESIAN_POINT('Ctrl Pts',(16.8841144424798,-19.981418490006,-18.8264131304831));
#79763=CARTESIAN_POINT('Ctrl Pts',(16.8887460996236,-19.9896979517452,-18.8258476330491));
#79764=CARTESIAN_POINT('Ctrl Pts',(16.8956954529312,-20.001926834905,-18.8250040381805));
#79765=CARTESIAN_POINT('Ctrl Pts',(16.8979706403711,-20.0059004488585,-18.8247286065803));
#79766=CARTESIAN_POINT('Ctrl Pts',(16.9020434470251,-20.0129603879956,-18.8242368412663));
#79767=CARTESIAN_POINT('Ctrl Pts',(16.9038360027987,-20.0160495759128,-18.8240208358815));
#79768=CARTESIAN_POINT('Ctrl Pts',(16.9077088762315,-20.0226851241615,-18.8235550636621));
#79769=CARTESIAN_POINT('Ctrl Pts',(16.9097916793271,-20.0262299129979,-18.8233051407437));
#79770=CARTESIAN_POINT('Ctrl Pts',(16.9155744862816,-20.03600653928,-18.8226128459874));
#79771=CARTESIAN_POINT('Ctrl Pts',(16.9192961456524,-20.042225409565,-18.8221690997641));
#79772=CARTESIAN_POINT('Ctrl Pts',(16.9399459765362,-20.0763324587598,-18.8197172739954));
#79773=CARTESIAN_POINT('Ctrl Pts',(16.9574841480153,-20.1038439448968,-18.8176726554272));
#79774=CARTESIAN_POINT('Ctrl Pts',(17.0662168518925,-20.2660155521638,-18.805264759139));
#79775=CARTESIAN_POINT('Ctrl Pts',(17.172044238368,-20.3902043111935,-18.7943129840949));
#79776=CARTESIAN_POINT('Ctrl Pts',(17.3764984374317,-20.5806550935415,-18.7760619146059));
#79777=CARTESIAN_POINT('Ctrl Pts',(17.468403734541,-20.6530590231472,-18.7686227995385));
#79778=CARTESIAN_POINT('Ctrl Pts',(17.5777443467583,-20.7254052103008,-18.7606173482261));
#79779=CARTESIAN_POINT('Ctrl Pts',(17.5897407312338,-20.733169255611,-18.759749393334));
#79780=CARTESIAN_POINT('Ctrl Pts',(17.608958805573,-20.7453328714826,-18.7583751118294));
#79781=CARTESIAN_POINT('Ctrl Pts',(17.6161296709972,-20.7498115607239,-18.7578658573277));
#79782=CARTESIAN_POINT('Ctrl Pts',(17.6288239836027,-20.7576346977653,-18.7569704863235));
#79783=CARTESIAN_POINT('Ctrl Pts',(17.6343362262835,-20.7609970357085,-18.7565837137265));
#79784=CARTESIAN_POINT('Ctrl Pts',(17.6457691779259,-20.7678992983185,-18.7557856437207));
#79785=CARTESIAN_POINT('Ctrl Pts',(17.6516919854971,-20.7714356122765,-18.7553744817097));
#79786=CARTESIAN_POINT('Ctrl Pts',(17.6669394830321,-20.7804385918038,-18.754321758977));
#79787=CARTESIAN_POINT('Ctrl Pts',(17.6762890194396,-20.7858629499039,-18.7536817396316));
#79788=CARTESIAN_POINT('Ctrl Pts',(17.7154849428461,-20.8082039297598,-18.7510209714955));
#79789=CARTESIAN_POINT('Ctrl Pts',(17.7456997525526,-20.8244659591105,-18.749023753765));
#79790=CARTESIAN_POINT('Ctrl Pts',(17.8254447527903,-20.8649174860893,-18.7438793930431));
#79791=CARTESIAN_POINT('Ctrl Pts',(17.8755486531456,-20.8879204209889,-18.7407716447346));
#79792=CARTESIAN_POINT('Ctrl Pts',(18.0275779349079,-20.950653079891,-18.7316269039943));
#79793=CARTESIAN_POINT('Ctrl Pts',(18.1317423616883,-20.9844696524625,-18.7257386398546));
#79794=CARTESIAN_POINT('Ctrl Pts',(18.2827853275708,-21.0208672103745,-18.7172798203817));
#79795=CARTESIAN_POINT('Ctrl Pts',(18.3278563773501,-21.0301851048364,-18.7147638438892));
#79796=CARTESIAN_POINT('Ctrl Pts',(18.3949976153116,-21.0417980794796,-18.7109848781702));
#79797=CARTESIAN_POINT('Ctrl Pts',(18.4168587241051,-21.0452271719869,-18.7097495995151));
#79798=CARTESIAN_POINT('Ctrl Pts',(18.4897489455725,-21.0554925537055,-18.7056033962618));
#79799=CARTESIAN_POINT('Ctrl Pts',(18.5409694612286,-21.0608095662436,-18.7026452989099));
#79800=CARTESIAN_POINT('Ctrl Pts',(18.6009481606497,-21.0648324230259,-18.699077409215));
#79801=CARTESIAN_POINT('Ctrl Pts',(18.6095715145293,-21.0653577988538,-18.6985619360271));
#79802=CARTESIAN_POINT('Ctrl Pts',(18.6226567844534,-21.0660746513971,-18.6977756223819));
#79803=CARTESIAN_POINT('Ctrl Pts',(18.627116608313,-21.0663048226472,-18.6975068987528));
#79804=CARTESIAN_POINT('Ctrl Pts',(18.635135790304,-21.0666932548656,-18.6970223501101));
#79805=CARTESIAN_POINT('Ctrl Pts',(18.638694845575,-21.0668566432179,-18.6968068152881));
#79806=CARTESIAN_POINT('Ctrl Pts',(18.6464438424468,-21.0671927818179,-18.6963364759373));
#79807=CARTESIAN_POINT('Ctrl Pts',(18.650633836454,-21.0673620652389,-18.6960814852294));
#79808=CARTESIAN_POINT('Ctrl Pts',(18.662442174101,-21.067804005904,-18.6953610256101));
#79809=CARTESIAN_POINT('Ctrl Pts',(18.6700614367456,-21.0680479602122,-18.6948939967365));
#79810=CARTESIAN_POINT('Ctrl Pts',(18.7164072015587,-21.0692813272485,-18.6920407641863));
#79811=CARTESIAN_POINT('Ctrl Pts',(18.7551509430224,-21.0692486686368,-18.6896028519034));
#79812=CARTESIAN_POINT('Ctrl Pts',(18.8845131907873,-21.0655888262614,-18.681333952897));
#79813=CARTESIAN_POINT('Ctrl Pts',(18.974893523719,-21.0572031384328,-18.6753490967955));
#79814=CARTESIAN_POINT('Ctrl Pts',(19.1307471124744,-21.0325733814219,-18.6649220879059));
#79815=CARTESIAN_POINT('Ctrl Pts',(19.1965089919515,-21.0189494052263,-18.660487687018));
#79816=CARTESIAN_POINT('Ctrl Pts',(19.3726487719311,-20.9736293677325,-18.6486167199407));
#79817=CARTESIAN_POINT('Ctrl Pts',(19.4812879707059,-20.9360427574739,-18.6413128955223));
#79818=CARTESIAN_POINT('Ctrl Pts',(19.5994120513845,-20.8840854817969,-18.6334336638356));
#79819=CARTESIAN_POINT('Ctrl Pts',(19.6124064128512,-20.8782124797467,-18.6325675373782));
#79820=CARTESIAN_POINT('Ctrl Pts',(19.6330013965653,-20.8686525038525,-18.6311955947777));
#79821=CARTESIAN_POINT('Ctrl Pts',(19.6406408312576,-20.8650506365165,-18.6306868662307));
#79822=CARTESIAN_POINT('Ctrl Pts',(19.6540808683156,-20.8586152906548,-18.6297921068231));
#79823=CARTESIAN_POINT('Ctrl Pts',(19.6598904104937,-20.8558008351681,-18.629405422689));
#79824=CARTESIAN_POINT('Ctrl Pts',(19.6718843373592,-20.849922443605,-18.6286072350012));
#79825=CARTESIAN_POINT('Ctrl Pts',(19.6780668011357,-20.8468547461299,-18.6281958683257));
#79826=CARTESIAN_POINT('Ctrl Pts',(19.6939073019939,-20.8388980227925,-18.6271419992971));
#79827=CARTESIAN_POINT('Ctrl Pts',(19.7035431180672,-20.8339650171127,-18.6265010449154));
#79828=CARTESIAN_POINT('Ctrl Pts',(19.7436812226261,-20.8130264287069,-18.6238311729969));
#79829=CARTESIAN_POINT('Ctrl Pts',(19.7738294151995,-20.7963509768782,-18.6218259925375));
#79830=CARTESIAN_POINT('Ctrl Pts',(19.8513829875248,-20.750948394958,-18.61665646518));
#79831=CARTESIAN_POINT('Ctrl Pts',(19.8980917830871,-20.7210819776976,-18.6135320203849));
#79832=CARTESIAN_POINT('Ctrl Pts',(20.0335300057599,-20.6267907518905,-18.6043581632974));
#79833=CARTESIAN_POINT('Ctrl Pts',(20.1184857249567,-20.5572733191734,-18.5984573789497));
#79834=CARTESIAN_POINT('Ctrl Pts',(20.2426992191399,-20.4384047657141,-18.5890955320172));
#79835=CARTESIAN_POINT('Ctrl Pts',(20.2857958590893,-20.3933539943715,-18.5856824603306));
#79836=CARTESIAN_POINT('Ctrl Pts',(20.3639012475826,-20.3041377457612,-18.5790298356332));
#79837=CARTESIAN_POINT('Ctrl Pts',(20.399256256701,-20.2603481887809,-18.5758080523372));
#79838=CARTESIAN_POINT('Ctrl Pts',(20.438092472647,-20.2081193643591,-18.5719465619758));
#79839=CARTESIAN_POINT('Ctrl Pts',(20.4433182777822,-20.2009988118277,-18.5714197176639));
#79840=CARTESIAN_POINT('Ctrl Pts',(20.4511432992934,-20.1901955442262,-18.5706194554781));
#79841=CARTESIAN_POINT('Ctrl Pts',(20.4537756370564,-20.1865367849415,-18.5703482686789));
#79842=CARTESIAN_POINT('Ctrl Pts',(20.4584693906847,-20.1799686618464,-18.5698610983468));
#79843=CARTESIAN_POINT('Ctrl Pts',(20.4605351578184,-20.1770624728657,-18.5696454190418));
#79844=CARTESIAN_POINT('Ctrl Pts',(20.4649961607319,-20.1707528917966,-18.5691768850585));
#79845=CARTESIAN_POINT('Ctrl Pts',(20.4673886733092,-20.1673476976924,-18.5689238557573));
#79846=CARTESIAN_POINT('Ctrl Pts',(20.4740516026647,-20.1578048464379,-18.5682143389553));
#79847=CARTESIAN_POINT('Ctrl Pts',(20.4782995167663,-20.151651657609,-18.5677563648471));
#79848=CARTESIAN_POINT('Ctrl Pts',(20.5029286578228,-20.1155684793673,-18.5650685572634));
#79849=CARTESIAN_POINT('Ctrl Pts',(20.5225705690355,-20.0851439269181,-18.5627935961272));
#79850=CARTESIAN_POINT('Ctrl Pts',(20.5834967394197,-19.9852383128982,-18.5553330064697));
#79851=CARTESIAN_POINT('Ctrl Pts',(20.6215844027536,-19.9138955167407,-18.5500224958001));
#79852=CARTESIAN_POINT('Ctrl Pts',(20.7329517894314,-19.6730640035333,-18.5325028904051));
#79853=CARTESIAN_POINT('Ctrl Pts',(20.7881900015719,-19.4961251383215,-18.5203482820602));
#79854=CARTESIAN_POINT('Ctrl Pts',(20.823578394119,-19.292359193749,-18.5076281932193));
#79855=CARTESIAN_POINT('Ctrl Pts',(20.8270341481658,-19.2704185288717,-18.5062730881744));
#79856=CARTESIAN_POINT('Ctrl Pts',(20.8313307743985,-19.2400354945448,-18.5044159785995));
#79857=CARTESIAN_POINT('Ctrl Pts',(20.8324670567682,-19.2316369758864,-18.503904672391));
#79858=CARTESIAN_POINT('Ctrl Pts',(20.8343321428887,-19.2171997031284,-18.5030291612216));
#79859=CARTESIAN_POINT('Ctrl Pts',(20.8350854048173,-19.2111642642324,-18.5026641873878));
#79860=CARTESIAN_POINT('Ctrl Pts',(20.8365834849316,-19.1987250499832,-18.5019140550896));
#79861=CARTESIAN_POINT('Ctrl Pts',(20.8373250833411,-19.1923209449959,-18.5015290019172));
#79862=CARTESIAN_POINT('Ctrl Pts',(20.8389808961183,-19.1774270115935,-18.5006360895484));
#79863=CARTESIAN_POINT('Ctrl Pts',(20.8398730268565,-19.168934802639,-18.5001289310879));
#79864=CARTESIAN_POINT('Ctrl Pts',(20.8425572207124,-19.1418051705631,-18.4985148331182));
#79865=CARTESIAN_POINT('Ctrl Pts',(20.8441534603499,-19.1231489494608,-18.4974140497023));
#79866=CARTESIAN_POINT('Ctrl Pts',(20.8472975481736,-19.0796086255421,-18.4948649144028));
#79867=CARTESIAN_POINT('Ctrl Pts',(20.8486537667875,-19.054713233871,-18.4934225047331));
#79868=CARTESIAN_POINT('Ctrl Pts',(20.8518757022942,-18.967099821794,-18.4883928473224));
#79869=CARTESIAN_POINT('Ctrl Pts',(20.8513931145288,-18.9043262670549,-18.4848740890824));
#79870=CARTESIAN_POINT('Ctrl Pts',(20.8428720657502,-18.7410579587601,-18.4758356516143));
#79871=CARTESIAN_POINT('Ctrl Pts',(20.8304470317565,-18.6409562042584,-18.4704107149107));
#79872=CARTESIAN_POINT('Ctrl Pts',(20.7965003148142,-18.4689423211722,-18.4608584099424));
#79873=CARTESIAN_POINT('Ctrl Pts',(20.778202868702,-18.3965853635209,-18.4567643522567));
#79874=CARTESIAN_POINT('Ctrl Pts',(20.7434988088597,-18.2845993373892,-18.4501073430232));
#79875=CARTESIAN_POINT('Ctrl Pts',(20.7296422710282,-18.2442426404533,-18.4476401718042));
#79876=CARTESIAN_POINT('Ctrl Pts',(20.7119384163549,-18.1973448132485,-18.4446622154976));
#79877=CARTESIAN_POINT('Ctrl Pts',(20.7092625937099,-18.1903685195962,-18.4442162996176));
#79878=CARTESIAN_POINT('Ctrl Pts',(20.7048754146731,-18.1791090807788,-18.4434916390452));
#79879=CARTESIAN_POINT('Ctrl Pts',(20.7031868665043,-18.1748170376021,-18.443214228184));
#79880=CARTESIAN_POINT('Ctrl Pts',(20.7001646590617,-18.1672081079149,-18.4427202904085));
#79881=CARTESIAN_POINT('Ctrl Pts',(20.6988366100738,-18.1638890459291,-18.4425041030383));
#79882=CARTESIAN_POINT('Ctrl Pts',(20.6959712249961,-18.156780132217,-18.4420394824604));
#79883=CARTESIAN_POINT('Ctrl Pts',(20.6944313352032,-18.1529914236201,-18.4417909012787));
#79884=CARTESIAN_POINT('Ctrl Pts',(20.690169542193,-18.1425922974893,-18.4411060081735));
#79885=CARTESIAN_POINT('Ctrl Pts',(20.6874251472724,-18.135991239428,-18.4406683688955));
#79886=CARTESIAN_POINT('Ctrl Pts',(20.6725197096794,-18.1006454991603,-18.4383099641676));
#79887=CARTESIAN_POINT('Ctrl Pts',(20.6597582143494,-18.0721601217494,-18.4363558007127));
#79888=CARTESIAN_POINT('Ctrl Pts',(20.5760966198343,-17.8959633301123,-18.4239771898663));
#79889=CARTESIAN_POINT('Ctrl Pts',(20.4888791166918,-17.7566203763466,-18.4129410329578));
#79890=CARTESIAN_POINT('Ctrl Pts',(20.3132340903315,-17.537279171229,-18.3945838729834));
#79891=CARTESIAN_POINT('Ctrl Pts',(20.2325273192082,-17.4520536403855,-18.3871198485398));
#79892=CARTESIAN_POINT('Ctrl Pts',(20.1345136163129,-17.364405931851,-18.3790912181555));
#79893=CARTESIAN_POINT('Ctrl Pts',(20.1237621753973,-17.3549857776881,-18.3782229636172));
#79894=CARTESIAN_POINT('Ctrl Pts',(20.106499878153,-17.3401673208972,-18.3768482988525));
#79895=CARTESIAN_POINT('Ctrl Pts',(20.1000508048977,-17.3346980174894,-18.3763389581962));
#79896=CARTESIAN_POINT('Ctrl Pts',(20.0886196633919,-17.3251206991501,-18.3754434869755));
#79897=CARTESIAN_POINT('Ctrl Pts',(20.0836512779953,-17.3209965906778,-18.3750566998546));
#79898=CARTESIAN_POINT('Ctrl Pts',(20.0733366261643,-17.3125141117848,-18.3742586489582));
#79899=CARTESIAN_POINT('Ctrl Pts',(20.0679877660476,-17.3081590047671,-18.3738475203385));
#79900=CARTESIAN_POINT('Ctrl Pts',(20.0542045866659,-17.2970481506091,-18.3727949846699));
#79901=CARTESIAN_POINT('Ctrl Pts',(20.0457395867717,-17.290330647359,-18.3721551179221));
#79902=CARTESIAN_POINT('Ctrl Pts',(20.0102055714285,-17.2625729574387,-18.3694958325998));
#79903=CARTESIAN_POINT('Ctrl Pts',(19.9826780098854,-17.2421263740964,-18.3674999116233));
#79904=CARTESIAN_POINT('Ctrl Pts',(19.9096807218189,-17.1906098513979,-18.362359645393));
#79905=CARTESIAN_POINT('Ctrl Pts',(19.8634732909611,-17.1606286972659,-18.3592546126373));
#79906=CARTESIAN_POINT('Ctrl Pts',(19.727837858173,-17.079960403585,-18.3504794197238));
#79907=CARTESIAN_POINT('Ctrl Pts',(19.6358199211269,-17.0339364658272,-18.3449341285276));
#79908=CARTESIAN_POINT('Ctrl Pts',(19.4803896648853,-16.9698636977147,-18.3357918249254));
#79909=CARTESIAN_POINT('Ctrl Pts',(19.4188372419515,-16.9477647244043,-18.3322228016808));
#79910=CARTESIAN_POINT('Ctrl Pts',(19.2986437188813,-16.9107961091291,-18.3251901395197));
#79911=CARTESIAN_POINT('Ctrl Pts',(19.2401953705464,-16.8955222643694,-18.3217421064812));
#79912=CARTESIAN_POINT('Ctrl Pts',(19.1724048409849,-16.8808720943795,-18.3176284568805));
#79913=CARTESIAN_POINT('Ctrl Pts',(19.1636175382026,-16.8790315076044,-18.317093039572));
#79914=CARTESIAN_POINT('Ctrl Pts',(19.1503711548645,-16.8763447640996,-18.3162822750475));
#79915=CARTESIAN_POINT('Ctrl Pts',(19.1459204975999,-16.8754569352647,-18.316009246889));
#79916=CARTESIAN_POINT('Ctrl Pts',(19.1379657000894,-16.8738966713928,-18.3155200946242));
#79917=CARTESIAN_POINT('Ctrl Pts',(19.1344626835415,-16.8732187777328,-18.3153042852115));
#79918=CARTESIAN_POINT('Ctrl Pts',(19.1268921048169,-16.8717735875005,-18.3148370007428));
#79919=CARTESIAN_POINT('Ctrl Pts',(19.1228240583786,-16.8710093743036,-18.3145853593082));
#79920=CARTESIAN_POINT('Ctrl Pts',(19.1115023629221,-16.8689168652911,-18.3138835525874));
#79921=CARTESIAN_POINT('Ctrl Pts',(19.1042440573122,-16.8676145475311,-18.3134319514192));
#79922=CARTESIAN_POINT('Ctrl Pts',(19.0640934201704,-16.8606268706243,-18.3109251497323));
#79923=CARTESIAN_POINT('Ctrl Pts',(19.0310789275326,-16.8556825015567,-18.3088317579333));
#79924=CARTESIAN_POINT('Ctrl Pts',(18.8373260946397,-16.8313339153715,-18.2964120106022));
#79925=CARTESIAN_POINT('Ctrl Pts',(18.6749075199446,-16.8296406854287,-18.2855109424445));
#79926=CARTESIAN_POINT('Ctrl Pts',(18.3979805757313,-16.858591214453,-18.2673255206477));
#79927=CARTESIAN_POINT('Ctrl Pts',(18.283261350022,-16.880258746877,-18.2599031165561));
#79928=CARTESIAN_POINT('Ctrl Pts',(18.1571215227772,-16.9150649736418,-18.2519132263159));
#79929=CARTESIAN_POINT('Ctrl Pts',(18.1433890974706,-16.9190042162842,-18.251045479298));
#79930=CARTESIAN_POINT('Ctrl Pts',(18.1215956177038,-16.9254952916182,-18.2496714636791));
#79931=CARTESIAN_POINT('Ctrl Pts',(18.1135083425481,-16.927956876245,-18.2491622689517));
#79932=CARTESIAN_POINT('Ctrl Pts',(18.0992705550748,-16.9323838932443,-18.2482669674717));
#79933=CARTESIAN_POINT('Ctrl Pts',(18.0931139241121,-16.93432913336,-18.2478802049454));
#79934=CARTESIAN_POINT('Ctrl Pts',(18.0803978464947,-16.9384109619467,-18.2470821216522));
#79935=CARTESIAN_POINT('Ctrl Pts',(18.0738397439389,-16.9405515101588,-18.2466709364509));
#79936=CARTESIAN_POINT('Ctrl Pts',(18.057031618539,-16.9461286979084,-18.2456180838121));
#79937=CARTESIAN_POINT('Ctrl Pts',(18.0467971646687,-16.9496118908345,-18.2449779584978));
#79938=CARTESIAN_POINT('Ctrl Pts',(18.0047965984569,-16.964266302249,-18.2423544795766));
#79939=CARTESIAN_POINT('Ctrl Pts',(17.9732714908691,-16.9761166088163,-18.2403936915787));
#79940=CARTESIAN_POINT('Ctrl Pts',(17.8919727295616,-17.0089112646876,-18.2353480281249));
#79941=CARTESIAN_POINT('Ctrl Pts',(17.8426929771977,-17.0310168764147,-18.2323009029342));
#79942=CARTESIAN_POINT('Ctrl Pts',(17.6803077428662,-17.1114547002125,-18.2222154692447));
#79943=CARTESIAN_POINT('Ctrl Pts',(17.5716302494621,-17.1780858783338,-18.2154056647421));
#79944=CARTESIAN_POINT('Ctrl Pts',(17.3877165003719,-17.3150422530441,-18.2028664152522));
#79945=CARTESIAN_POINT('Ctrl Pts',(17.3103691808172,-17.3818472560374,-18.1971988908188));
#79946=CARTESIAN_POINT('Ctrl Pts',(17.2312944835982,-17.4608061670488,-18.1905785117495));
#79947=CARTESIAN_POINT('Ctrl Pts',(17.224484104867,-17.4677006128363,-18.1900010107411));
#79948=CARTESIAN_POINT('Ctrl Pts',(17.2144982268397,-17.4779495618229,-18.1891429143673));
#79949=CARTESIAN_POINT('Ctrl Pts',(17.2112858742483,-17.4812682014599,-18.1888651196395));
#79950=CARTESIAN_POINT('Ctrl Pts',(17.2056059778469,-17.4871745843698,-18.1883707584947));
#79951=CARTESIAN_POINT('Ctrl Pts',(17.2031341027769,-17.4897580946576,-18.188154533796));
#79952=CARTESIAN_POINT('Ctrl Pts',(17.1978517445306,-17.4953070915276,-18.1876901273039));
#79953=CARTESIAN_POINT('Ctrl Pts',(17.1950433396807,-17.4982744105637,-18.1874417990732));
#79954=CARTESIAN_POINT('Ctrl Pts',(17.1892976820677,-17.504380495982,-18.1869308558748));
#79955=CARTESIAN_POINT('Ctrl Pts',(17.1863613664049,-17.5075201148841,-18.1866681727624));
#79956=CARTESIAN_POINT('Ctrl Pts',(17.1729077089025,-17.5219933826711,-18.185457478628));
#79957=CARTESIAN_POINT('Ctrl Pts',(17.1625054854867,-17.5334327559568,-18.1845012563713));
#79958=CARTESIAN_POINT('Ctrl Pts',(17.0941974976145,-17.6102247657089,-18.1780928140918));
#79959=CARTESIAN_POINT('Ctrl Pts',(17.0402626620495,-17.6789863629095,-18.1724082029247));
#79960=CARTESIAN_POINT('Ctrl Pts',(16.9494514377864,-17.8107861005604,-18.1618725522541));
#79961=CARTESIAN_POINT('Ctrl Pts',(16.9112865552785,-17.8727879806763,-18.157046709732));
#79962=CARTESIAN_POINT('Ctrl Pts',(16.87410699438,-17.9408078058736,-18.1519487847017));
#79963=CARTESIAN_POINT('Ctrl Pts',(16.8718386494663,-17.9449911864191,-18.151636005868));
#79964=CARTESIAN_POINT('Ctrl Pts',(16.8058494279297,-18.0676768142243,-18.1424856031553));
#79965=CARTESIAN_POINT('Ctrl Pts',(16.7535466437575,-18.1919945354638,-18.1338552605409));
#79966=CARTESIAN_POINT('Ctrl Pts',(16.7086937510272,-18.3355002086818,-18.1246738660042));
#79967=CARTESIAN_POINT('Ctrl Pts',(16.7041601067162,-18.3505954576644,-18.1237169459198));
#79968=CARTESIAN_POINT('Ctrl Pts',(16.6975600327991,-18.373496400646,-18.1222782755559));
#79969=CARTESIAN_POINT('Ctrl Pts',(16.6953690585521,-18.381265348987,-18.1217924773275));
#79970=CARTESIAN_POINT('Ctrl Pts',(16.691524469894,-18.3952024733846,-18.1209249582957));
#79971=CARTESIAN_POINT('Ctrl Pts',(16.6898542383013,-18.4013659263714,-18.1205427012609));
#79972=CARTESIAN_POINT('Ctrl Pts',(16.6863713131255,-18.4144528128727,-18.119733955102));
#79973=CARTESIAN_POINT('Ctrl Pts',(16.6845657850165,-18.4213780836742,-18.1193077023673));
#79974=CARTESIAN_POINT('Ctrl Pts',(16.6809624106011,-18.4354919538744,-18.1184424202491));
#79975=CARTESIAN_POINT('Ctrl Pts',(16.6791671181644,-18.4426811067311,-18.1180034781013));
#79976=CARTESIAN_POINT('Ctrl Pts',(16.6747876919857,-18.4606184102313,-18.1169126994108));
#79977=CARTESIAN_POINT('Ctrl Pts',(16.6722499088619,-18.4713777316691,-18.1162623476298));
#79978=CARTESIAN_POINT('Ctrl Pts',(16.6345655716992,-18.6369395762027,-18.1063131404208));
#79979=CARTESIAN_POINT('Ctrl Pts',(16.6168549652036,-18.7951908614192,-18.0976369962091));
#79980=CARTESIAN_POINT('Ctrl Pts',(16.6170008943745,-18.9539459653064,-18.0890147266704));
#79981=CARTESIAN_POINT('Ctrl Pts',(16.6170008942677,-18.9539458490376,-18.0890147329851));
#79982=CARTESIAN_POINT('Ctrl Pts',(16.617132245813,-19.0968506163556,-18.0812533231527));
#79983=CARTESIAN_POINT('Ctrl Pts',(16.6317330753476,-19.2393602546854,-18.0735574166762));
#79984=CARTESIAN_POINT('Ctrl Pts',(16.6625404198842,-19.3888517284755,-18.0645862748028));
#79985=CARTESIAN_POINT('Ctrl Pts',(16.6645760527504,-19.3983952772006,-18.0640094873609));
#79986=CARTESIAN_POINT('Ctrl Pts',(16.6678828636037,-19.4133895330032,-18.0630963762149));
#79987=CARTESIAN_POINT('Ctrl Pts',(16.669109829536,-19.4188499810754,-18.0627624050525));
#79988=CARTESIAN_POINT('Ctrl Pts',(16.6714750735612,-19.4291844290826,-18.0621274827003));
#79989=CARTESIAN_POINT('Ctrl Pts',(16.6726090155973,-19.4340593944653,-18.061826773435));
#79990=CARTESIAN_POINT('Ctrl Pts',(16.6745952714028,-19.4424633975876,-18.0613062272276));
#79991=CARTESIAN_POINT('Ctrl Pts',(16.6754394037885,-19.4459943847055,-18.0610868599088));
#79992=CARTESIAN_POINT('Ctrl Pts',(16.6770955964153,-19.4528442359433,-18.0606600010243));
#79993=CARTESIAN_POINT('Ctrl Pts',(16.6779066098708,-19.456163311683,-18.0604525759641));
#79994=CARTESIAN_POINT('Ctrl Pts',(16.6801205638094,-19.4651297326649,-18.0598906479025));
#79995=CARTESIAN_POINT('Ctrl Pts',(16.681538747412,-19.4707732315171,-18.0595352792088));
#79996=CARTESIAN_POINT('Ctrl Pts',(16.6869136685068,-19.4917950548166,-18.0582054256839));
#79997=CARTESIAN_POINT('Ctrl Pts',(16.691020011754,-19.5071341126097,-18.0572228373783));
#79998=CARTESIAN_POINT('Ctrl Pts',(16.7100014012788,-19.574973688845,-18.0528271902886));
#79999=CARTESIAN_POINT('Ctrl Pts',(16.7267229156432,-19.626906712487,-18.0493291599082));
#80000=CARTESIAN_POINT('Ctrl Pts',(16.7454193872878,-19.6781102855251,-18.0457833417799));
#80001=CARTESIAN_POINT('Origin',(18.734,-18.952,0.));
#80002=CARTESIAN_POINT('',(16.7454194498739,-19.6781104569281,-17.2426989690604));
#80003=CARTESIAN_POINT('',(16.745419450228,-19.6781104578977,-17.467776498566));
#80004=CARTESIAN_POINT('',(16.7454194499637,-19.6781104571739,0.));
#80005=CARTESIAN_POINT('Ctrl Pts',(16.745419450228,-19.6781104578977,-17.467776498566));
#80006=CARTESIAN_POINT('Ctrl Pts',(16.7278145373555,-19.6298963233431,-17.4710694417504));
#80007=CARTESIAN_POINT('Ctrl Pts',(16.7119674247689,-19.5810538475648,-17.4743159728977));
#80008=CARTESIAN_POINT('Ctrl Pts',(16.6884846842029,-19.4985720493969,-17.479647127548));
#80009=CARTESIAN_POINT('Ctrl Pts',(16.6798675447131,-19.4652387232586,-17.4817614672596));
#80010=CARTESIAN_POINT('Ctrl Pts',(16.669614458812,-19.421167833389,-17.484506134469));
#80011=CARTESIAN_POINT('Ctrl Pts',(16.6672430096864,-19.4106084041471,-17.4851599772679));
#80012=CARTESIAN_POINT('Ctrl Pts',(16.6634921056292,-19.3932863961265,-17.4862264942702));
#80013=CARTESIAN_POINT('Ctrl Pts',(16.6620645843557,-19.3865345316673,-17.4866407035569));
#80014=CARTESIAN_POINT('Ctrl Pts',(16.6593656416203,-19.3734533816376,-17.4874403333963));
#80015=CARTESIAN_POINT('Ctrl Pts',(16.6580901071281,-19.3671250317248,-17.4878258815601));
#80016=CARTESIAN_POINT('Ctrl Pts',(16.65521237201,-19.3525026263704,-17.4887137982358));
#80017=CARTESIAN_POINT('Ctrl Pts',(16.6536308201122,-19.3442045825099,-17.4892155031073));
#80018=CARTESIAN_POINT('Ctrl Pts',(16.649512270004,-19.3218694008198,-17.4905601871931));
#80019=CARTESIAN_POINT('Ctrl Pts',(16.6470673784447,-19.3078155675167,-17.4914002383051));
#80020=CARTESIAN_POINT('Ctrl Pts',(16.626190687621,-19.1801846309213,-17.4989769015963));
#80021=CARTESIAN_POINT('Ctrl Pts',(16.6169037092795,-19.065299216771,-17.5054071035181));
#80022=CARTESIAN_POINT('Ctrl Pts',(16.6171578062868,-18.7639639400357,-17.5219135265107));
#80023=CARTESIAN_POINT('Ctrl Pts',(16.6418924521979,-18.578581011756,-17.5316811112538));
#80024=CARTESIAN_POINT('Ctrl Pts',(16.694256245899,-18.3851344243615,-17.5434580684037));
#80025=CARTESIAN_POINT('Ctrl Pts',(16.6981093688863,-18.3714481272867,-17.5443004579815));
#80026=CARTESIAN_POINT('Ctrl Pts',(16.7036607297581,-18.3524648719532,-17.5454829971989));
#80027=CARTESIAN_POINT('Ctrl Pts',(16.7052425223522,-18.347133884778,-17.5458166422803));
#80028=CARTESIAN_POINT('Ctrl Pts',(16.7078156428536,-18.3385855522126,-17.5463542432883));
#80029=CARTESIAN_POINT('Ctrl Pts',(16.7087936868813,-18.3353641894629,-17.5465574266642));
#80030=CARTESIAN_POINT('Ctrl Pts',(16.7108530776938,-18.3286389672065,-17.5469828783114));
#80031=CARTESIAN_POINT('Ctrl Pts',(16.7119358447885,-18.3251355825079,-17.5472052320709));
#80032=CARTESIAN_POINT('Ctrl Pts',(16.7145777280571,-18.3166656110929,-17.5477445271499));
#80033=CARTESIAN_POINT('Ctrl Pts',(16.716146066486,-18.3117019445417,-17.5480620046195));
#80034=CARTESIAN_POINT('Ctrl Pts',(16.7216994320505,-18.294349029513,-17.5491768005403));
#80035=CARTESIAN_POINT('Ctrl Pts',(16.7257802907857,-18.2819910784939,-17.5499794650986));
#80036=CARTESIAN_POINT('Ctrl Pts',(16.7505712486492,-18.209179030544,-17.5547573500665));
#80037=CARTESIAN_POINT('Ctrl Pts',(16.7738944055408,-18.1496552434907,-17.5588615632688));
#80038=CARTESIAN_POINT('Ctrl Pts',(16.8760922808093,-17.9200048733331,-17.5752528705611));
#80039=CARTESIAN_POINT('Ctrl Pts',(16.9747462057869,-17.7595736626754,-17.5878515521336));
#80040=CARTESIAN_POINT('Ctrl Pts',(17.128654570568,-17.5708067306473,-17.6032548870418));
#80041=CARTESIAN_POINT('Ctrl Pts',(17.1657757998303,-17.528798475539,-17.6067354248861));
#80042=CARTESIAN_POINT('Ctrl Pts',(17.2128425128144,-17.4796163269227,-17.6108793336885));
#80043=CARTESIAN_POINT('Ctrl Pts',(17.2212358738615,-17.4709940953485,-17.611608568766));
#80044=CARTESIAN_POINT('Ctrl Pts',(17.2352366791693,-17.4568547317422,-17.6128091676919));
#80045=CARTESIAN_POINT('Ctrl Pts',(17.2408020912742,-17.451296540604,-17.6132823608392));
#80046=CARTESIAN_POINT('Ctrl Pts',(17.2509287698957,-17.4412951081666,-17.6141361329356));
#80047=CARTESIAN_POINT('Ctrl Pts',(17.2554793306571,-17.4368412045365,-17.61451718038));
#80048=CARTESIAN_POINT('Ctrl Pts',(17.2652853707379,-17.4273296962544,-17.6153327738553));
#80049=CARTESIAN_POINT('Ctrl Pts',(17.2705470436209,-17.4222785731252,-17.6157670343438));
#80050=CARTESIAN_POINT('Ctrl Pts',(17.2849677572284,-17.4085774181892,-17.6169481634482));
#80051=CARTESIAN_POINT('Ctrl Pts',(17.2941781651148,-17.3999817008966,-17.6176926871672));
#80052=CARTESIAN_POINT('Ctrl Pts',(17.343313531804,-17.354939438352,-17.6216137829902));
#80053=CARTESIAN_POINT('Ctrl Pts',(17.3845488252999,-17.3199480580817,-17.6247285100711));
#80054=CARTESIAN_POINT('Ctrl Pts',(17.5775455933136,-17.1684969047962,-17.6386249859452));
#80055=CARTESIAN_POINT('Ctrl Pts',(17.7433014241674,-17.0713669327261,-17.6486491865709));
#80056=CARTESIAN_POINT('Ctrl Pts',(17.9351116018922,-16.9914541473783,-17.6602002585299));
#80057=CARTESIAN_POINT('Ctrl Pts',(17.9504572506331,-16.9852708745889,-17.6611247414616));
#80058=CARTESIAN_POINT('Ctrl Pts',(18.0154371536849,-16.959969520619,-17.6650468852495));
#80059=CARTESIAN_POINT('Ctrl Pts',(18.0657061740732,-16.9425472520998,-17.668099243892));
#80060=CARTESIAN_POINT('Ctrl Pts',(18.1249048980915,-16.9244970945919,-17.6717720142836));
#80061=CARTESIAN_POINT('Ctrl Pts',(18.1332522419629,-16.9220081281144,-17.6722916800794));
#80062=CARTESIAN_POINT('Ctrl Pts',(18.145916687653,-16.9183168637882,-17.6730831390944));
#80063=CARTESIAN_POINT('Ctrl Pts',(18.1502227551509,-16.9170766087342,-17.6733527736882));
#80064=CARTESIAN_POINT('Ctrl Pts',(18.1579604175239,-16.9148745496692,-17.6738382878472));
#80065=CARTESIAN_POINT('Ctrl Pts',(18.1613905293181,-16.913907731541,-17.6740538720244));
#80066=CARTESIAN_POINT('Ctrl Pts',(18.1688506107295,-16.9118253377499,-17.6745235251855));
#80067=CARTESIAN_POINT('Ctrl Pts',(18.1728813964128,-16.9107130538088,-17.6747777760013));
#80068=CARTESIAN_POINT('Ctrl Pts',(18.184216700423,-16.9076212194275,-17.6754941009582));
#80069=CARTESIAN_POINT('Ctrl Pts',(18.191528491049,-16.9056689092541,-17.6759577071562));
#80070=CARTESIAN_POINT('Ctrl Pts',(18.235382845567,-16.8942109794016,-17.6787468819658));
#80071=CARTESIAN_POINT('Ctrl Pts',(18.2721615201621,-16.8856458361256,-17.6811215559806));
#80072=CARTESIAN_POINT('Ctrl Pts',(18.3941300914431,-16.8606600724104,-17.6890699536874));
#80073=CARTESIAN_POINT('Ctrl Pts',(18.4800978884145,-16.848491964533,-17.6947857651894));
#80074=CARTESIAN_POINT('Ctrl Pts',(18.7418263909396,-16.8277264202923,-17.7121324653516));
#80075=CARTESIAN_POINT('Ctrl Pts',(18.9181758879456,-16.8357055199715,-17.7236768034007));
#80076=CARTESIAN_POINT('Ctrl Pts',(19.1141647727758,-16.8692875610003,-17.7359157672763));
#80077=CARTESIAN_POINT('Ctrl Pts',(19.1367352434748,-16.8735340400004,-17.7373176331889));
#80078=CARTESIAN_POINT('Ctrl Pts',(19.1685801250482,-16.8800636690634,-17.7392854451132));
#80079=CARTESIAN_POINT('Ctrl Pts',(19.1779144317484,-16.8820434723188,-17.7398610149612));
#80080=CARTESIAN_POINT('Ctrl Pts',(19.1930628252236,-16.8853636227724,-17.7407931707343));
#80081=CARTESIAN_POINT('Ctrl Pts',(19.1988851156082,-16.8866655419519,-17.7411509825978));
#80082=CARTESIAN_POINT('Ctrl Pts',(19.2110637386624,-16.8894429056283,-17.741898486785));
#80083=CARTESIAN_POINT('Ctrl Pts',(19.2174189182583,-16.890923162706,-17.7422880201902));
#80084=CARTESIAN_POINT('Ctrl Pts',(19.232526468667,-16.8945157537857,-17.7432127893382));
#80085=CARTESIAN_POINT('Ctrl Pts',(19.241272453318,-16.8966545970809,-17.7437471659618));
#80086=CARTESIAN_POINT('Ctrl Pts',(19.2707150346374,-16.9040542037183,-17.7455429722428));
#80087=CARTESIAN_POINT('Ctrl Pts',(19.2913460269346,-16.9095724080665,-17.7467960910483));
#80088=CARTESIAN_POINT('Ctrl Pts',(19.403356258191,-16.9413556345067,-17.7535761794883));
#80089=CARTESIAN_POINT('Ctrl Pts',(19.4929752629715,-16.9734429080522,-17.7589088427267));
#80090=CARTESIAN_POINT('Ctrl Pts',(19.7363115714171,-17.079545364619,-17.7735134467975));
#80091=CARTESIAN_POINT('Ctrl Pts',(19.8836711959582,-17.1662343191764,-17.7824759839761));
#80092=CARTESIAN_POINT('Ctrl Pts',(20.048552498187,-17.2921746194202,-17.794322069814));
#80093=CARTESIAN_POINT('Ctrl Pts',(20.0774690342639,-17.3154917838281,-17.7964789767863));
#80094=CARTESIAN_POINT('Ctrl Pts',(20.1112115357397,-17.3441975548522,-17.7991126283722));
#80095=CARTESIAN_POINT('Ctrl Pts',(20.1166440942714,-17.3488669356307,-17.7995403718011));
#80096=CARTESIAN_POINT('Ctrl Pts',(20.1254647929601,-17.3565266686795,-17.8002411863204));
#80097=CARTESIAN_POINT('Ctrl Pts',(20.1288672920435,-17.359500499931,-17.8005130626462));
#80098=CARTESIAN_POINT('Ctrl Pts',(20.1349380775842,-17.3648408325228,-17.8010009730552));
#80099=CARTESIAN_POINT('Ctrl Pts',(20.1376099281236,-17.3672032024468,-17.8012166989892));
#80100=CARTESIAN_POINT('Ctrl Pts',(20.1433802634822,-17.372331198733,-17.8016847555476));
#80101=CARTESIAN_POINT('Ctrl Pts',(20.1464765407044,-17.3750991565526,-17.8019372576699));
#80102=CARTESIAN_POINT('Ctrl Pts',(20.1550952620772,-17.382849726684,-17.8026438425883));
#80103=CARTESIAN_POINT('Ctrl Pts',(20.1605995582269,-17.3878523021026,-17.8030993926092));
#80104=CARTESIAN_POINT('Ctrl Pts',(20.1922720582496,-17.4169440815917,-17.8057450338897));
#80105=CARTESIAN_POINT('Ctrl Pts',(20.2178545770922,-17.4416592049688,-17.8079786492476));
#80106=CARTESIAN_POINT('Ctrl Pts',(20.2978229168524,-17.5229095085538,-17.8152428688612));
#80107=CARTESIAN_POINT('Ctrl Pts',(20.3496920383832,-17.5818250753066,-17.8203916877443));
#80108=CARTESIAN_POINT('Ctrl Pts',(20.5144698303587,-17.7913882872951,-17.8379874255252));
#80109=CARTESIAN_POINT('Ctrl Pts',(20.6105594130797,-17.9541794143467,-17.8503964698286));
#80110=CARTESIAN_POINT('Ctrl Pts',(20.6923693512098,-18.1476646945847,-17.8633118362426));
#80111=CARTESIAN_POINT('Ctrl Pts',(20.7005616519169,-18.1679074515319,-17.864643826459));
#80112=CARTESIAN_POINT('Ctrl Pts',(20.711475681688,-18.196123186614,-17.8664745615214));
#80113=CARTESIAN_POINT('Ctrl Pts',(20.7144650189755,-18.2039905478562,-17.8669822677787));
#80114=CARTESIAN_POINT('Ctrl Pts',(20.7195283612208,-18.2175594434026,-17.867853241419));
#80115=CARTESIAN_POINT('Ctrl Pts',(20.7216249019649,-18.2232524067499,-17.8682172598299));
#80116=CARTESIAN_POINT('Ctrl Pts',(20.7259016343792,-18.2350212369487,-17.8689669111436));
#80117=CARTESIAN_POINT('Ctrl Pts',(20.7280785686044,-18.2410982266401,-17.8693524322109));
#80118=CARTESIAN_POINT('Ctrl Pts',(20.7330881853936,-18.2552868259416,-17.8702489391956));
#80119=CARTESIAN_POINT('Ctrl Pts',(20.7358993622759,-18.263405949397,-17.870759206552));
#80120=CARTESIAN_POINT('Ctrl Pts',(20.7447721193394,-18.2895455084089,-17.8723933985687));
#80121=CARTESIAN_POINT('Ctrl Pts',(20.7506405097874,-18.3076308833396,-17.8735109456384));
#80122=CARTESIAN_POINT('Ctrl Pts',(20.7789096093923,-18.3989227851026,-17.8790898709617));
#80123=CARTESIAN_POINT('Ctrl Pts',(20.7975726116513,-18.4732311752088,-17.8834281140622));
#80124=CARTESIAN_POINT('Ctrl Pts',(20.8331227192317,-18.656278848617,-17.8937908286963));
#80125=CARTESIAN_POINT('Ctrl Pts',(20.8456426825138,-18.7656315762455,-17.8997059276357));
#80126=CARTESIAN_POINT('Ctrl Pts',(20.8521618575798,-18.945835922279,-17.909526728321));
#80127=CARTESIAN_POINT('Ctrl Pts',(20.8511947689397,-19.0162867885636,-17.9133874850769));
#80128=CARTESIAN_POINT('Ctrl Pts',(20.843675002066,-19.1343596947872,-17.9200725876549));
#80129=CARTESIAN_POINT('Ctrl Pts',(20.8390088837037,-19.1820445862877,-17.922832093884));
#80130=CARTESIAN_POINT('Ctrl Pts',(20.831716743104,-19.2371898066608,-17.9261346949096));
#80131=CARTESIAN_POINT('Ctrl Pts',(20.8306613725614,-19.2448478185067,-17.9265958377179));
#80132=CARTESIAN_POINT('Ctrl Pts',(20.8289055491562,-19.257092223195,-17.9273374258822));
#80133=CARTESIAN_POINT('Ctrl Pts',(20.8282319091574,-19.2616824732989,-17.927616397696));
#80134=CARTESIAN_POINT('Ctrl Pts',(20.8270106633001,-19.2698179221795,-17.9281125924166));
#80135=CARTESIAN_POINT('Ctrl Pts',(20.8264691291266,-19.2733639865203,-17.9283294695038));
#80136=CARTESIAN_POINT('Ctrl Pts',(20.8253005432132,-19.2808879047706,-17.9287909196289));
#80137=CARTESIAN_POINT('Ctrl Pts',(20.8246711637287,-19.2848652887816,-17.9290356167509));
#80138=CARTESIAN_POINT('Ctrl Pts',(20.8229381171665,-19.295618498979,-17.9296991881539));
#80139=CARTESIAN_POINT('Ctrl Pts',(20.8218128431955,-19.302390723329,-17.9301192582767));
#80140=CARTESIAN_POINT('Ctrl Pts',(20.8160132847415,-19.3362740501696,-17.9322314104331));
#80141=CARTESIAN_POINT('Ctrl Pts',(20.8108440047118,-19.363296336031,-17.9339493125006));
#80142=CARTESIAN_POINT('Ctrl Pts',(20.7942858840615,-19.4415566561962,-17.9390072848292));
#80143=CARTESIAN_POINT('Ctrl Pts',(20.7815167274972,-19.4924795555058,-17.9424020358221));
#80144=CARTESIAN_POINT('Ctrl Pts',(20.7277878889936,-19.6773314205922,-17.9549904834507));
#80145=CARTESIAN_POINT('Ctrl Pts',(20.6754578583809,-19.8075943668165,-17.9643539487579));
#80146=CARTESIAN_POINT('Ctrl Pts',(20.5673798944559,-20.0146138090563,-17.9794560317214));
#80147=CARTESIAN_POINT('Ctrl Pts',(20.5186649396223,-20.0945432683055,-17.9853563567417));
#80148=CARTESIAN_POINT('Ctrl Pts',(20.4568674936831,-20.1822874562478,-17.991905285481));
#80149=CARTESIAN_POINT('Ctrl Pts',(20.4488069964224,-20.1934977265337,-17.9927435596222));
#80150=CARTESIAN_POINT('Ctrl Pts',(20.435717997427,-20.2113307651203,-17.994079817909));
#80151=CARTESIAN_POINT('Ctrl Pts',(20.4307592501047,-20.2180040161901,-17.9945804831779));
#80152=CARTESIAN_POINT('Ctrl Pts',(20.421893141664,-20.229789945465,-17.9954659117261));
#80153=CARTESIAN_POINT('Ctrl Pts',(20.4180015635411,-20.2349143142924,-17.9958512852074));
#80154=CARTESIAN_POINT('Ctrl Pts',(20.4098529272256,-20.245543346032,-17.9966515072384));
#80155=CARTESIAN_POINT('Ctrl Pts',(20.4055919646096,-20.251044928932,-17.9970661954092));
#80156=CARTESIAN_POINT('Ctrl Pts',(20.394474131314,-20.2652545458578,-17.9981386135188));
#80157=CARTESIAN_POINT('Ctrl Pts',(20.3875758074244,-20.2739299902588,-17.9987946873923));
#80158=CARTESIAN_POINT('Ctrl Pts',(20.3574947852159,-20.31115644722,-18.0016161870161));
#80159=CARTESIAN_POINT('Ctrl Pts',(20.3336375784294,-20.3391558758331,-18.0037542983399));
#80160=CARTESIAN_POINT('Ctrl Pts',(20.2685087528343,-20.4116764973964,-18.0093503088328));
#80161=CARTESIAN_POINT('Ctrl Pts',(20.2260306807968,-20.4550694791138,-18.0127591017667));
#80162=CARTESIAN_POINT('Ctrl Pts',(20.0631393871247,-20.6077484814625,-18.0251198802547));
#80163=CARTESIAN_POINT('Ctrl Pts',(19.9321358206603,-20.7048772656731,-18.0336927930378));
#80164=CARTESIAN_POINT('Ctrl Pts',(19.7414663596128,-20.8147968027434,-18.0460280754051));
#80165=CARTESIAN_POINT('Ctrl Pts',(19.6904661444035,-20.8414897878346,-18.0493202579872));
#80166=CARTESIAN_POINT('Ctrl Pts',(19.6304186964888,-20.8698637522312,-18.0532601877973));
#80167=CARTESIAN_POINT('Ctrl Pts',(19.6223664241616,-20.8736068645068,-18.0537898204125));
#80168=CARTESIAN_POINT('Ctrl Pts',(19.6101826138716,-20.8791775825208,-18.0545934997434));
#80169=CARTESIAN_POINT('Ctrl Pts',(19.6060682677586,-20.8810428566834,-18.0548652869437));
#80170=CARTESIAN_POINT('Ctrl Pts',(19.5986951356964,-20.8843571206202,-18.0553531015523));
#80171=CARTESIAN_POINT('Ctrl Pts',(19.5954386311095,-20.8858110569209,-18.0555688213183));
#80172=CARTESIAN_POINT('Ctrl Pts',(19.5883808065901,-20.8889408083918,-18.0560369389422));
#80173=CARTESIAN_POINT('Ctrl Pts',(19.5845782755089,-20.8906136423822,-18.0562895086996));
#80174=CARTESIAN_POINT('Ctrl Pts',(19.5739491837222,-20.8952523684646,-18.0569964695375));
#80175=CARTESIAN_POINT('Ctrl Pts',(19.5671119469399,-20.8981934330538,-18.0574523303214));
#80176=CARTESIAN_POINT('Ctrl Pts',(19.5274374274844,-20.915012208453,-18.0601033296458));
#80177=CARTESIAN_POINT('Ctrl Pts',(19.4942713519237,-20.9280938757247,-18.0623421943833));
#80178=CARTESIAN_POINT('Ctrl Pts',(19.3868409024943,-20.9673628503226,-18.0696311619156));
#80179=CARTESIAN_POINT('Ctrl Pts',(19.3114428514005,-20.9902459971906,-18.0748003112139));
#80180=CARTESIAN_POINT('Ctrl Pts',(19.0525855787614,-21.0532906141568,-18.0923861963261));
#80181=CARTESIAN_POINT('Ctrl Pts',(18.8650793089506,-21.073265143475,-18.1047628427769));
#80182=CARTESIAN_POINT('Ctrl Pts',(18.6554961582511,-21.0676571365953,-18.1176535355759));
#80183=CARTESIAN_POINT('Ctrl Pts',(18.6336283222385,-21.0667325021242,-18.1189886028542));
#80184=CARTESIAN_POINT('Ctrl Pts',(18.6033682105101,-21.0649825598461,-18.1208228563401));
#80185=CARTESIAN_POINT('Ctrl Pts',(18.5949612134311,-21.0644460186423,-18.1213310488727));
#80186=CARTESIAN_POINT('Ctrl Pts',(18.5805035304397,-21.063436634994,-18.1222026350934));
#80187=CARTESIAN_POINT('Ctrl Pts',(18.5744513113502,-21.0629879314921,-18.122566782213));
#80188=CARTESIAN_POINT('Ctrl Pts',(18.5619669217578,-21.062008358501,-18.1233164963825));
#80189=CARTESIAN_POINT('Ctrl Pts',(18.5555350756361,-21.0614740873377,-18.1237019524874));
#80190=CARTESIAN_POINT('Ctrl Pts',(18.5405539541994,-21.0601606490404,-18.1245979655291));
#80191=CARTESIAN_POINT('Ctrl Pts',(18.5320067359999,-21.0593588729516,-18.125107806354));
#80192=CARTESIAN_POINT('Ctrl Pts',(18.5045860860872,-21.0566183055288,-18.1267392318985));
#80193=CARTESIAN_POINT('Ctrl Pts',(18.4857334213134,-21.05447775171,-18.1278544697676));
#80194=CARTESIAN_POINT('Ctrl Pts',(18.3912626732096,-21.0424629752717,-18.1334139694499));
#80195=CARTESIAN_POINT('Ctrl Pts',(18.3161842460222,-21.0287609633748,-18.1377360970775));
#80196=CARTESIAN_POINT('Ctrl Pts',(18.0773748424344,-20.9716985198246,-18.1513837359916));
#80197=CARTESIAN_POINT('Ctrl Pts',(17.9180734980709,-20.9127641214443,-18.1602911163621));
#80198=CARTESIAN_POINT('Ctrl Pts',(17.7613194130465,-20.832327021385,-18.1701569555515));
#80199=CARTESIAN_POINT('Ctrl Pts',(17.7551562201155,-20.8291260172312,-18.1705468248623));
#80200=CARTESIAN_POINT('Ctrl Pts',(17.7028138526511,-20.8016128586891,-18.1738755930327));
#80201=CARTESIAN_POINT('Ctrl Pts',(17.6575364368848,-20.7756331414273,-18.1768726740398));
#80202=CARTESIAN_POINT('Ctrl Pts',(17.6059737175145,-20.7434574106965,-18.18047977821));
#80203=CARTESIAN_POINT('Ctrl Pts',(17.5987062147721,-20.7388606447802,-18.1809928107255));
#80204=CARTESIAN_POINT('Ctrl Pts',(17.5877557857993,-20.7318406208264,-18.1817731799165));
#80205=CARTESIAN_POINT('Ctrl Pts',(17.5840519913075,-20.7294498616357,-18.182038408293));
#80206=CARTESIAN_POINT('Ctrl Pts',(17.5775081618246,-20.7251968762569,-18.1825093356745));
#80207=CARTESIAN_POINT('Ctrl Pts',(17.5746651128291,-20.7233393669585,-18.1827147185618));
#80208=CARTESIAN_POINT('Ctrl Pts',(17.5718041261608,-20.7214602995117,-18.1829221940531));
#80209=CARTESIAN_POINT('Ctrl Pts',(17.5717817453369,-20.7214455994025,-18.182923817134));
#80210=CARTESIAN_POINT('Ctrl Pts',(17.5717374603198,-20.7214165110405,-18.1829270288269));
#80211=CARTESIAN_POINT('Ctrl Pts',(17.5717155564107,-20.7214021230001,-18.1829286174163));
#80212=CARTESIAN_POINT('Ctrl Pts',(17.5716721963381,-20.7213736398775,-18.1829317622151));
#80213=CARTESIAN_POINT('Ctrl Pts',(17.5716507400462,-20.7213595447347,-18.1829333184319));
#80214=CARTESIAN_POINT('Ctrl Pts',(17.5716082477229,-20.7213316294216,-18.1829364004733));
#80215=CARTESIAN_POINT('Ctrl Pts',(17.5715872117662,-20.721317809322,-18.1829379262908));
#80216=CARTESIAN_POINT('Ctrl Pts',(17.5715455349472,-20.721290427626,-18.1829409493539));
#80217=CARTESIAN_POINT('Ctrl Pts',(17.5715248941418,-20.7212768660868,-18.1829424465938));
#80218=CARTESIAN_POINT('Ctrl Pts',(17.5714839844136,-20.72124998632,-18.1829454141805));
#80219=CARTESIAN_POINT('Ctrl Pts',(17.5714637154324,-20.7212366680724,-18.1829468845301));
#80220=CARTESIAN_POINT('Ctrl Pts',(17.5714235280464,-20.7212102609435,-18.1829497998776));
#80221=CARTESIAN_POINT('Ctrl Pts',(17.5714036093988,-20.7211971719198,-18.1829512448917));
#80222=CARTESIAN_POINT('Ctrl Pts',(17.5713641022553,-20.7211712098677,-18.1829541110458));
#80223=CARTESIAN_POINT('Ctrl Pts',(17.571344513777,-20.7211583368667,-18.1829555321832));
#80224=CARTESIAN_POINT('Ctrl Pts',(17.5713056478953,-20.7211327943702,-18.1829583519641));
#80225=CARTESIAN_POINT('Ctrl Pts',(17.5712863706823,-20.7211201250144,-18.1829597505926));
#80226=CARTESIAN_POINT('Ctrl Pts',(17.5712481100679,-20.7210949785061,-18.1829625266047));
#80227=CARTESIAN_POINT('Ctrl Pts',(17.5712291266373,-20.7210825013479,-18.1829639039894));
#80228=CARTESIAN_POINT('Ctrl Pts',(17.5711914372614,-20.7210577285445,-18.1829666386951));
#80229=CARTESIAN_POINT('Ctrl Pts',(17.5711727312304,-20.7210454328555,-18.1829679960213));
#80230=CARTESIAN_POINT('Ctrl Pts',(17.5711355812659,-20.7210210129135,-18.1829706917238));
#80231=CARTESIAN_POINT('Ctrl Pts',(17.5711171372815,-20.7210088886387,-18.1829720301027));
#80232=CARTESIAN_POINT('Ctrl Pts',(17.571080496686,-20.720984801881,-18.1829746889762));
#80233=CARTESIAN_POINT('Ctrl Pts',(17.5710623001659,-20.7209728394689,-18.1829760094633));
#80234=CARTESIAN_POINT('Ctrl Pts',(17.5710261413792,-20.7209490678442,-18.1829786335024));
#80235=CARTESIAN_POINT('Ctrl Pts',(17.5710081789585,-20.7209372585405,-18.1829799370648));
#80236=CARTESIAN_POINT('Ctrl Pts',(17.5709724748682,-20.7209137842859,-18.1829825282321));
#80237=CARTESIAN_POINT('Ctrl Pts',(17.5709547334959,-20.72090211954,-18.1829838158146));
#80238=CARTESIAN_POINT('Ctrl Pts',(17.5709194597347,-20.7208789266924,-18.1829863758739));
#80239=CARTESIAN_POINT('Ctrl Pts',(17.5709019273821,-20.7208673986234,-18.1829876483473));
#80240=CARTESIAN_POINT('Ctrl Pts',(17.5708670602951,-20.7208444716831,-18.182990179011));
#80241=CARTESIAN_POINT('Ctrl Pts',(17.5708497255287,-20.720833072799,-18.182991437203));
#80242=CARTESIAN_POINT('Ctrl Pts',(17.5708152429612,-20.7208103972483,-18.1829939400751));
#80243=CARTESIAN_POINT('Ctrl Pts',(17.5707980950534,-20.7207991205193,-18.1829951847623));
#80244=CARTESIAN_POINT('Ctrl Pts',(17.5707639756402,-20.7207766823554,-18.1829976613898));
#80245=CARTESIAN_POINT('Ctrl Pts',(17.570747004238,-20.7207655209957,-18.1829988933219));
#80246=CARTESIAN_POINT('Ctrl Pts',(17.5707132280953,-20.7207433071862,-18.1830013451445));
#80247=CARTESIAN_POINT('Ctrl Pts',(17.5706964233892,-20.7207322547658,-18.1830025650319));
#80248=CARTESIAN_POINT('Ctrl Pts',(17.5706629717341,-20.7207102529986,-18.1830049934098));
#80249=CARTESIAN_POINT('Ctrl Pts',(17.5706463245488,-20.7206993035027,-18.1830062019169));
#80250=CARTESIAN_POINT('Ctrl Pts',(17.5706131793865,-20.7206775019807,-18.1830086081533));
#80251=CARTESIAN_POINT('Ctrl Pts',(17.5705966811634,-20.7206666497986,-18.1830098059));
#80252=CARTESIAN_POINT('Ctrl Pts',(17.570563824197,-20.7206450365227,-18.1830121913202));
#80253=CARTESIAN_POINT('Ctrl Pts',(17.5705474659792,-20.72063427578,-18.1830133789553));
#80254=CARTESIAN_POINT('Ctrl Pts',(17.5705148823415,-20.7206128410041,-18.1830157446361));
#80255=CARTESIAN_POINT('Ctrl Pts',(17.570498656574,-20.7206021667472,-18.1830169227067));
#80256=CARTESIAN_POINT('Ctrl Pts',(17.5669733594806,-20.7182829510758,-18.1832728822284));
#80257=CARTESIAN_POINT('Ctrl Pts',(17.5634712015733,-20.7159639946129,-18.1835283658869));
#80258=CARTESIAN_POINT('Ctrl Pts',(17.5533745623766,-20.7092351892539,-18.1842683500758));
#80259=CARTESIAN_POINT('Ctrl Pts',(17.5467980218839,-20.7047987314328,-18.1847545907038));
#80260=CARTESIAN_POINT('Ctrl Pts',(17.5031777922752,-20.6750149220107,-18.1880072092336));
#80261=CARTESIAN_POINT('Ctrl Pts',(17.4669261534767,-20.6485338013872,-18.190843091036));
#80262=CARTESIAN_POINT('Ctrl Pts',(17.3376286846866,-20.5476280480046,-18.2013741625363));
#80263=CARTESIAN_POINT('Ctrl Pts',(17.2500690229898,-20.4665391393246,-18.2093154794288));
#80264=CARTESIAN_POINT('Ctrl Pts',(17.070835538936,-20.2700066449078,-18.2268361359592));
#80265=CARTESIAN_POINT('Ctrl Pts',(16.983418077119,-20.1514729917286,-18.2363012277721));
#80266=CARTESIAN_POINT('Ctrl Pts',(16.9017510066727,-20.0125448676335,-18.2461406433001));
#80267=CARTESIAN_POINT('Ctrl Pts',(16.8946583767629,-20.000195687072,-18.2470056080363));
#80268=CARTESIAN_POINT('Ctrl Pts',(16.8835611924874,-19.9804145364375,-18.2483760643911));
#80269=CARTESIAN_POINT('Ctrl Pts',(16.8794756432188,-19.9730287226287,-18.2488844585938));
#80270=CARTESIAN_POINT('Ctrl Pts',(16.8723439638226,-19.959952113074,-18.2497788294476));
#80271=CARTESIAN_POINT('Ctrl Pts',(16.8692795042379,-19.9542714868748,-18.2501654575796));
#80272=CARTESIAN_POINT('Ctrl Pts',(16.862991058598,-19.9424858426101,-18.2509637211513));
#80273=CARTESIAN_POINT('Ctrl Pts',(16.8597708575872,-19.9363788837048,-18.2513752187681));
#80274=CARTESIAN_POINT('Ctrl Pts',(16.8515737311609,-19.920647376848,-18.2524298207301));
#80275=CARTESIAN_POINT('Ctrl Pts',(16.846640677324,-19.9110001001063,-18.2530713728825));
#80276=CARTESIAN_POINT('Ctrl Pts',(16.8262952097781,-19.8704465919449,-18.2557470804528));
#80277=CARTESIAN_POINT('Ctrl Pts',(16.8115656643136,-19.8392024201524,-18.2577573662174));
#80278=CARTESIAN_POINT('Ctrl Pts',(16.778791499888,-19.7650288552953,-18.2624217793942));
#80279=CARTESIAN_POINT('Ctrl Pts',(16.7613864427332,-19.7218388607945,-18.2650549637422));
#80280=CARTESIAN_POINT('Ctrl Pts',(16.745419450845,-19.6781104595875,-18.2676549380821));
#80281=CARTESIAN_POINT('Ctrl Pts',(16.7454193872878,-19.6781102855251,-18.0457833417799));
#80282=CARTESIAN_POINT('Ctrl Pts',(16.7693936118093,-19.74376791225,-18.0412365887061));
#80283=CARTESIAN_POINT('Ctrl Pts',(16.7966152266407,-19.8082261759475,-18.0366121350535));
#80284=CARTESIAN_POINT('Ctrl Pts',(16.8578701043261,-19.9353018072534,-18.0272902389871));
#80285=CARTESIAN_POINT('Ctrl Pts',(16.8919573327061,-19.9977654881651,-18.0226009975555));
#80286=CARTESIAN_POINT('Ctrl Pts',(16.9780524348281,-20.1382131432663,-18.0118976631239));
#80287=CARTESIAN_POINT('Ctrl Pts',(17.0322252502904,-20.2147035228647,-18.0059486028066));
#80288=CARTESIAN_POINT('Ctrl Pts',(17.1052039057518,-20.3044787334957,-17.9988355474707));
#80289=CARTESIAN_POINT('Ctrl Pts',(17.1193830444339,-20.3213748886869,-17.9974902752154));
#80290=CARTESIAN_POINT('Ctrl Pts',(17.1384824928375,-20.3434249922963,-17.9957252654999));
#80291=CARTESIAN_POINT('Ctrl Pts',(17.1431680433609,-20.3487796220301,-17.9952959019302));
#80292=CARTESIAN_POINT('Ctrl Pts',(17.1524850363611,-20.3593193498321,-17.9944492379624));
#80293=CARTESIAN_POINT('Ctrl Pts',(17.1571151993546,-20.3645054548259,-17.9940318919085));
#80294=CARTESIAN_POINT('Ctrl Pts',(17.1660812176998,-20.3744489875953,-17.9932302181764));
#80295=CARTESIAN_POINT('Ctrl Pts',(17.1704133815653,-20.379209626602,-17.9928457417555));
#80296=CARTESIAN_POINT('Ctrl Pts',(17.1804002879802,-20.3900842427672,-17.9919659233094));
#80297=CARTESIAN_POINT('Ctrl Pts',(17.1860695534442,-20.3961847839294,-17.9914712059013));
#80298=CARTESIAN_POINT('Ctrl Pts',(17.201266138522,-20.4123451209219,-17.9901574964782));
#80299=CARTESIAN_POINT('Ctrl Pts',(17.2108565646309,-20.422345214983,-17.9893412226815));
#80300=CARTESIAN_POINT('Ctrl Pts',(17.2872013390473,-20.5004025426934,-17.9829410960019));
#80301=CARTESIAN_POINT('Ctrl Pts',(17.3583895325229,-20.5639788844936,-17.9775621476939));
#80302=CARTESIAN_POINT('Ctrl Pts',(17.5143262243304,-20.6853616863687,-17.9666495829469));
#80303=CARTESIAN_POINT('Ctrl Pts',(17.5994685176907,-20.7422473287287,-17.9611478091277));
#80304=CARTESIAN_POINT('Ctrl Pts',(17.7570931387863,-20.8317832892747,-17.9512617703116));
#80305=CARTESIAN_POINT('Ctrl Pts',(17.8279227704957,-20.8669293300417,-17.9469131895881));
#80306=CARTESIAN_POINT('Ctrl Pts',(17.9333381983799,-20.9120771349535,-17.9403514629299));
#80307=CARTESIAN_POINT('Ctrl Pts',(17.9664795984596,-20.9252900926776,-17.9382759520062));
#80308=CARTESIAN_POINT('Ctrl Pts',(18.0068870952703,-20.940228038729,-17.9357122556132));
#80309=CARTESIAN_POINT('Ctrl Pts',(18.0138508293981,-20.9427609295474,-17.9352692603445));
#80310=CARTESIAN_POINT('Ctrl Pts',(18.0247634647876,-20.9466653882889,-17.9345730132578));
#80311=CARTESIAN_POINT('Ctrl Pts',(18.0287034523018,-20.9480619362208,-17.934321219382));
#80312=CARTESIAN_POINT('Ctrl Pts',(18.0360102047989,-20.9506275159754,-17.9338534515313));
#80313=CARTESIAN_POINT('Ctrl Pts',(18.039375795226,-20.9517997188161,-17.933637668691));
#80314=CARTESIAN_POINT('Ctrl Pts',(18.0469814189056,-20.9544271683891,-17.9331493153539));
#80315=CARTESIAN_POINT('Ctrl Pts',(18.0512230996814,-20.9558774411146,-17.9328764568797));
#80316=CARTESIAN_POINT('Ctrl Pts',(18.0637275845528,-20.9601085370153,-17.9320706595235));
#80317=CARTESIAN_POINT('Ctrl Pts',(18.0720028802374,-20.9628517634983,-17.9315355850433));
#80318=CARTESIAN_POINT('Ctrl Pts',(18.1310095042004,-20.9820085073495,-17.9277086034642));
#80319=CARTESIAN_POINT('Ctrl Pts',(18.1823238144446,-20.9965499332094,-17.9243197205658));
#80320=CARTESIAN_POINT('Ctrl Pts',(18.2514714852123,-21.0133524250873,-17.9197208026075));
#80321=CARTESIAN_POINT('Ctrl Pts',(18.2688680759763,-21.0173473935484,-17.9185610543798));
#80322=CARTESIAN_POINT('Ctrl Pts',(18.4475858537301,-21.056015813411,-17.9066314229938));
#80323=CARTESIAN_POINT('Ctrl Pts',(18.6124100646995,-21.0719390599156,-17.8955614339438));
#80324=CARTESIAN_POINT('Ctrl Pts',(18.8531727896178,-21.0670009749237,-17.8801417825589));
#80325=CARTESIAN_POINT('Ctrl Pts',(18.9288029784438,-21.0613803171453,-17.8753960106413));
#80326=CARTESIAN_POINT('Ctrl Pts',(19.0178487259798,-21.0499310078119,-17.8699246123796));
#80327=CARTESIAN_POINT('Ctrl Pts',(19.0317029290583,-21.0480099220996,-17.86907660208));
#80328=CARTESIAN_POINT('Ctrl Pts',(19.0531996865828,-21.0448116425523,-17.8677656478585));
#80329=CARTESIAN_POINT('Ctrl Pts',(19.0608557934811,-21.0436295809423,-17.8672997081182));
#80330=CARTESIAN_POINT('Ctrl Pts',(19.0747857084879,-21.0414005250706,-17.8664536475409));
#80331=CARTESIAN_POINT('Ctrl Pts',(19.0810615885703,-21.0403672350382,-17.866073097295));
#80332=CARTESIAN_POINT('Ctrl Pts',(19.0946146228468,-21.0380730185192,-17.865252600454));
#80333=CARTESIAN_POINT('Ctrl Pts',(19.1018900448154,-21.0368022596519,-17.8648129713455));
#80334=CARTESIAN_POINT('Ctrl Pts',(19.1216341082358,-21.0332470970613,-17.8636220556546));
#80335=CARTESIAN_POINT('Ctrl Pts',(19.1340892478913,-21.0308887139837,-17.8628731273959));
#80336=CARTESIAN_POINT('Ctrl Pts',(19.1950019111816,-21.0187871780044,-17.8592210163664));
#80337=CARTESIAN_POINT('Ctrl Pts',(19.2431314240933,-21.0074604723946,-17.8563687029365));
#80338=CARTESIAN_POINT('Ctrl Pts',(19.3300587152406,-20.9837620051366,-17.8512511582915));
#80339=CARTESIAN_POINT('Ctrl Pts',(19.3689790980515,-20.9719367871477,-17.8489724874093));
#80340=CARTESIAN_POINT('Ctrl Pts',(19.5830361901105,-20.9001005188713,-17.8364468755194));
#80341=CARTESIAN_POINT('Ctrl Pts',(19.7500303845104,-20.8184476352614,-17.8267723700119));
#80342=CARTESIAN_POINT('Ctrl Pts',(19.9385731007309,-20.6933752742972,-17.8138977969149));
#80343=CARTESIAN_POINT('Ctrl Pts',(19.9722093725219,-20.6696208095459,-17.8115121651604));
#80344=CARTESIAN_POINT('Ctrl Pts',(20.0113290505122,-20.6402474956649,-17.8086027096268));
#80345=CARTESIAN_POINT('Ctrl Pts',(20.0175032145462,-20.63555831617,-17.8081394013585));
#80346=CARTESIAN_POINT('Ctrl Pts',(20.0269991210544,-20.6282637304151,-17.8074202076817));
#80347=CARTESIAN_POINT('Ctrl Pts',(20.0303391355034,-20.6256820683754,-17.8071659675805));
#80348=CARTESIAN_POINT('Ctrl Pts',(20.0364823399228,-20.6209042618402,-17.8066959451347));
#80349=CARTESIAN_POINT('Ctrl Pts',(20.039287719743,-20.6187110274869,-17.8064803686794));
#80350=CARTESIAN_POINT('Ctrl Pts',(20.0455716383609,-20.6137726899483,-17.8059953887306));
#80351=CARTESIAN_POINT('Ctrl Pts',(20.049047075152,-20.6110237565865,-17.8057257150846));
#80352=CARTESIAN_POINT('Ctrl Pts',(20.0578942383287,-20.6039807325387,-17.8050355826186));
#80353=CARTESIAN_POINT('Ctrl Pts',(20.0632536703179,-20.5996713786234,-17.8046140662291));
#80354=CARTESIAN_POINT('Ctrl Pts',(20.0940126448746,-20.5746912907569,-17.8021754183637));
#80355=CARTESIAN_POINT('Ctrl Pts',(20.1189493404682,-20.5534607304561,-17.8001214848639));
#80356=CARTESIAN_POINT('Ctrl Pts',(20.2722964420945,-20.4166436975308,-17.787052808929));
#80357=CARTESIAN_POINT('Ctrl Pts',(20.3866452805175,-20.2862799923726,-17.7753881239929));
#80358=CARTESIAN_POINT('Ctrl Pts',(20.538613230693,-20.0630879329642,-17.7578248716403));
#80359=CARTESIAN_POINT('Ctrl Pts',(20.5877451883144,-19.9790241345162,-17.7516410983881));
#80360=CARTESIAN_POINT('Ctrl Pts',(20.6405228267156,-19.8725035509622,-17.7443372880991));
#80361=CARTESIAN_POINT('Ctrl Pts',(20.6498208818888,-19.8529919416943,-17.7430197631765));
#80362=CARTESIAN_POINT('Ctrl Pts',(20.6625851614088,-19.8251151821034,-17.7411653993401));
#80363=CARTESIAN_POINT('Ctrl Pts',(20.666298799818,-19.8168654220279,-17.7406200579321));
#80364=CARTESIAN_POINT('Ctrl Pts',(20.6726029557417,-19.8026175766791,-17.7396840388364));
#80365=CARTESIAN_POINT('Ctrl Pts',(20.6752187780872,-19.7966308891183,-17.7392924973758));
#80366=CARTESIAN_POINT('Ctrl Pts',(20.6801667413029,-19.7851623506839,-17.7385457473988));
#80367=CARTESIAN_POINT('Ctrl Pts',(20.6825035346509,-19.779682586576,-17.7381903829529));
#80368=CARTESIAN_POINT('Ctrl Pts',(20.6885039127454,-19.7654454903334,-17.7372707866537));
#80369=CARTESIAN_POINT('Ctrl Pts',(20.6921318073627,-19.7566731884048,-17.7367077707049));
#80370=CARTESIAN_POINT('Ctrl Pts',(20.7042219197092,-19.726873117927,-17.7348070905714));
#80371=CARTESIAN_POINT('Ctrl Pts',(20.7124055777902,-19.7057335006389,-17.7334788098968));
#80372=CARTESIAN_POINT('Ctrl Pts',(20.782377154087,-19.515989610415,-17.7217234681205));
#80373=CARTESIAN_POINT('Ctrl Pts',(20.8228190666641,-19.3402970886071,-17.712088878132));
#80374=CARTESIAN_POINT('Ctrl Pts',(20.8489329988472,-19.0778304230901,-17.6977272841027));
#80375=CARTESIAN_POINT('Ctrl Pts',(20.8522629491512,-18.9936501035693,-17.6931104868366));
#80376=CARTESIAN_POINT('Ctrl Pts',(20.8498286810781,-18.8724118636735,-17.6861818769906));
#80377=CARTESIAN_POINT('Ctrl Pts',(20.8481091707749,-18.8353496038035,-17.6840257623756));
#80378=CARTESIAN_POINT('Ctrl Pts',(20.8448705662682,-18.7908443280256,-17.6813705740444));
#80379=CARTESIAN_POINT('Ctrl Pts',(20.8442840196782,-18.7833374654045,-17.6809204457278));
#80380=CARTESIAN_POINT('Ctrl Pts',(20.8433101782056,-18.7716753277115,-17.6802174105148));
#80381=CARTESIAN_POINT('Ctrl Pts',(20.8429506158881,-18.7675177125768,-17.6799660337094));
#80382=CARTESIAN_POINT('Ctrl Pts',(20.8422611386093,-18.7598108284493,-17.6794986428312));
#80383=CARTESIAN_POINT('Ctrl Pts',(20.8419345517853,-18.7562613195348,-17.6792828173551));
#80384=CARTESIAN_POINT('Ctrl Pts',(20.8411761378834,-18.7482405776633,-17.6787938551327));
#80385=CARTESIAN_POINT('Ctrl Pts',(20.8407390456659,-18.743769908845,-17.6785204272316));
#80386=CARTESIAN_POINT('Ctrl Pts',(20.8394074873847,-18.730583946111,-17.6777114216681));
#80387=CARTESIAN_POINT('Ctrl Pts',(20.8384731569533,-18.7218728994083,-17.677173683437));
#80388=CARTESIAN_POINT('Ctrl Pts',(20.831346153911,-18.6591026363319,-17.673276359708));
#80389=CARTESIAN_POINT('Ctrl Pts',(20.8231258686592,-18.6052987339085,-17.669815802896));
#80390=CARTESIAN_POINT('Ctrl Pts',(20.8079047420478,-18.5262173015384,-17.6646074650703));
#80391=CARTESIAN_POINT('Ctrl Pts',(20.8024914932381,-18.5006524003797,-17.6629045327568));
#80392=CARTESIAN_POINT('Ctrl Pts',(20.7656089183897,-18.341102404484,-17.6521791688563));
#80393=CARTESIAN_POINT('Ctrl Pts',(20.7216054697338,-18.210339866693,-17.6429844498354));
#80394=CARTESIAN_POINT('Ctrl Pts',(20.6398097258069,-18.0281895750498,-17.6300818320424));
#80395=CARTESIAN_POINT('Ctrl Pts',(20.6119240084307,-17.9727457059202,-17.6261358421616));
#80396=CARTESIAN_POINT('Ctrl Pts',(20.5634080540366,-17.8860026460309,-17.6199423725365));
#80397=CARTESIAN_POINT('Ctrl Pts',(20.544314439973,-17.8538897623401,-17.6176445784271));
#80398=CARTESIAN_POINT('Ctrl Pts',(20.5184327855038,-17.8128718941052,-17.6147011787904));
#80399=CARTESIAN_POINT('Ctrl Pts',(20.5124110952523,-17.8034934952971,-17.6140275929162));
#80400=CARTESIAN_POINT('Ctrl Pts',(20.5025023090888,-17.7883259934935,-17.6129371069797));
#80401=CARTESIAN_POINT('Ctrl Pts',(20.4986602376119,-17.7825078630994,-17.6125185368357));
#80402=CARTESIAN_POINT('Ctrl Pts',(20.4912197051231,-17.7713606590949,-17.6117160194871));
#80403=CARTESIAN_POINT('Ctrl Pts',(20.4876255756273,-17.7660287999786,-17.6113319154873));
#80404=CARTESIAN_POINT('Ctrl Pts',(20.4793454019425,-17.7538651755275,-17.6104550387788));
#80405=CARTESIAN_POINT('Ctrl Pts',(20.4746434182545,-17.7470443480522,-17.6099628764798));
#80406=CARTESIAN_POINT('Ctrl Pts',(20.4620560413474,-17.729012189554,-17.6086604336094));
#80407=CARTESIAN_POINT('Ctrl Pts',(20.454101518667,-17.717849423612,-17.6078527968192));
#80408=CARTESIAN_POINT('Ctrl Pts',(20.3933122321799,-17.6342719562811,-17.6017937214933));
#80409=CARTESIAN_POINT('Ctrl Pts',(20.3360310618835,-17.5651966353714,-17.5967220776201));
#80410=CARTESIAN_POINT('Ctrl Pts',(20.1788562727152,-17.3984432328899,-17.5840326092265));
#80411=CARTESIAN_POINT('Ctrl Pts',(20.0733814625243,-17.3066417416989,-17.5766122070599));
#80412=CARTESIAN_POINT('Ctrl Pts',(19.9141818591566,-17.1936004370378,-17.5658309436337));
#80413=CARTESIAN_POINT('Ctrl Pts',(19.867462249585,-17.1631286505904,-17.562707799087));
#80414=CARTESIAN_POINT('Ctrl Pts',(19.7950071468588,-17.1198500887044,-17.5578405708402));
#80415=CARTESIAN_POINT('Ctrl Pts',(19.7701220587053,-17.1056629885674,-17.5561647922503));
#80416=CARTESIAN_POINT('Ctrl Pts',(19.7388464650812,-17.0886640210807,-17.5540439634812));
#80417=CARTESIAN_POINT('Ctrl Pts',(19.7327184496974,-17.0853723338889,-17.553627725962));
#80418=CARTESIAN_POINT('Ctrl Pts',(19.7229997152573,-17.080213435689,-17.5529663267001));
#80419=CARTESIAN_POINT('Ctrl Pts',(19.7194196109493,-17.0783261839799,-17.552722415704));
#80420=CARTESIAN_POINT('Ctrl Pts',(19.7126599401845,-17.0747875564422,-17.5522613316506));
#80421=CARTESIAN_POINT('Ctrl Pts',(19.7094815854193,-17.0731339822743,-17.5520443003138));
#80422=CARTESIAN_POINT('Ctrl Pts',(19.7022086767756,-17.0693735999185,-17.5515471580382));
#80423=CARTESIAN_POINT('Ctrl Pts',(19.6981114417043,-17.0672720803474,-17.5512667192591));
#80424=CARTESIAN_POINT('Ctrl Pts',(19.6872225580158,-17.0617318426961,-17.5505205039179));
#80425=CARTESIAN_POINT('Ctrl Pts',(19.6804192335744,-17.0583163986691,-17.5500533296973));
#80426=CARTESIAN_POINT('Ctrl Pts',(19.6328430162482,-17.0347523286347,-17.5467805626035));
#80427=CARTESIAN_POINT('Ctrl Pts',(19.5914515921,-17.0158870143595,-17.5439039320113));
#80428=CARTESIAN_POINT('Ctrl Pts',(19.5442118732782,-16.9961681017593,-17.5406137141424));
#80429=CARTESIAN_POINT('Ctrl Pts',(19.5389264162691,-16.9939869364191,-17.5402454832081));
#80430=CARTESIAN_POINT('Ctrl Pts',(19.3878092937333,-16.9323402676795,-17.5297156380831));
#80431=CARTESIAN_POINT('Ctrl Pts',(19.2358034663099,-16.8893102486276,-17.5191256203768));
#80432=CARTESIAN_POINT('Ctrl Pts',(18.9788177328514,-16.8466825928729,-17.5022143684257));
#80433=CARTESIAN_POINT('Ctrl Pts',(18.876104813786,-16.8372638948765,-17.4956951972229));
#80434=CARTESIAN_POINT('Ctrl Pts',(18.7582952600754,-16.8350876255305,-17.4885096311951));
#80435=CARTESIAN_POINT('Ctrl Pts',(18.7434875798233,-16.8349694701884,-17.4876115069509));
#80436=CARTESIAN_POINT('Ctrl Pts',(18.7209109500846,-16.8350262097226,-17.4862496124459));
#80437=CARTESIAN_POINT('Ctrl Pts',(18.7131424099457,-16.8350884960878,-17.4857823308274));
#80438=CARTESIAN_POINT('Ctrl Pts',(18.69901349972,-16.8352795621371,-17.484934856235));
#80439=CARTESIAN_POINT('Ctrl Pts',(18.6926530595032,-16.8353942504218,-17.4845542266078));
#80440=CARTESIAN_POINT('Ctrl Pts',(18.678927403502,-16.8357036381158,-17.4837346976736));
#80441=CARTESIAN_POINT('Ctrl Pts',(18.6715624751479,-16.8359081211337,-17.483296109709));
#80442=CARTESIAN_POINT('Ctrl Pts',(18.6516067723349,-16.8365664545909,-17.4821107776325));
#80443=CARTESIAN_POINT('Ctrl Pts',(18.6390186128716,-16.8370942632281,-17.4813663544352));
#80444=CARTESIAN_POINT('Ctrl Pts',(18.577949934905,-16.8402011620293,-17.4777700543958));
#80445=CARTESIAN_POINT('Ctrl Pts',(18.5295609594839,-16.8443351392701,-17.4749671528917));
#80446=CARTESIAN_POINT('Ctrl Pts',(18.4408402304731,-16.8549994204974,-17.4698882870485));
#80447=CARTESIAN_POINT('Ctrl Pts',(18.4004743829692,-16.8610396968277,-17.467600608625));
#80448=CARTESIAN_POINT('Ctrl Pts',(18.2279671460885,-16.8919765050713,-17.4578738577562));
#80449=CARTESIAN_POINT('Ctrl Pts',(18.0981936187453,-16.9282619744091,-17.4507040359213));
#80450=CARTESIAN_POINT('Ctrl Pts',(17.9142079942015,-16.9991649604153,-17.4398677466165));
#80451=CARTESIAN_POINT('Ctrl Pts',(17.8567128028137,-17.0243097633019,-17.4363742109886));
#80452=CARTESIAN_POINT('Ctrl Pts',(17.7726606680223,-17.065608597365,-17.4309874974222));
#80453=CARTESIAN_POINT('Ctrl Pts',(17.7452021025995,-17.079855687701,-17.4291811158706));
#80454=CARTESIAN_POINT('Ctrl Pts',(17.7118128456444,-17.098119410001,-17.4269145457118));
#80455=CARTESIAN_POINT('Ctrl Pts',(17.7055759330753,-17.1015720074039,-17.4264881038169));
#80456=CARTESIAN_POINT('Ctrl Pts',(17.6957925209745,-17.1070525969064,-17.4258141574643));
#80457=CARTESIAN_POINT('Ctrl Pts',(17.6922341844883,-17.1090595032209,-17.4255679853148));
#80458=CARTESIAN_POINT('Ctrl Pts',(17.6855723009197,-17.1128422727838,-17.4251050888916));
#80459=CARTESIAN_POINT('Ctrl Pts',(17.6824674364376,-17.1146157035432,-17.424888520867));
#80460=CARTESIAN_POINT('Ctrl Pts',(17.6753618171657,-17.1186981875299,-17.4243910040629));
#80461=CARTESIAN_POINT('Ctrl Pts',(17.6713641284959,-17.1210124682511,-17.4241097204899));
#80462=CARTESIAN_POINT('Ctrl Pts',(17.6590006515957,-17.1282238707399,-17.4232356134878));
#80463=CARTESIAN_POINT('Ctrl Pts',(17.6506610396186,-17.1331653023303,-17.4226400250973));
#80464=CARTESIAN_POINT('Ctrl Pts',(17.5601832148601,-17.1876187224859,-17.4161155732146));
#80465=CARTESIAN_POINT('Ctrl Pts',(17.4814755037281,-17.2425950820262,-17.4098775435969));
#80466=CARTESIAN_POINT('Ctrl Pts',(17.3080589833185,-17.3821475748548,-17.3952245706541));
#80467=CARTESIAN_POINT('Ctrl Pts',(17.2166658688101,-17.4702962509117,-17.3867947967225));
#80468=CARTESIAN_POINT('Ctrl Pts',(17.0955502512068,-17.6101476027983,-17.3748732461246));
#80469=CARTESIAN_POINT('Ctrl Pts',(17.0592305945565,-17.6557616599507,-17.3711748626576));
#80470=CARTESIAN_POINT('Ctrl Pts',(17.0037578913632,-17.7316609561797,-17.3653244375874));
#80471=CARTESIAN_POINT('Ctrl Pts',(16.9834112147788,-17.7610322063367,-17.363128715548));
#80472=CARTESIAN_POINT('Ctrl Pts',(16.957800802189,-17.8000773821775,-17.3602956476176));
#80473=CARTESIAN_POINT('Ctrl Pts',(16.9518562852668,-17.809295709781,-17.3596328517881));
#80474=CARTESIAN_POINT('Ctrl Pts',(16.9422715547169,-17.8244157469037,-17.358555467737));
#80475=CARTESIAN_POINT('Ctrl Pts',(16.938588272585,-17.8302897877315,-17.3581392837314));
#80476=CARTESIAN_POINT('Ctrl Pts',(16.931537785762,-17.841657493327,-17.3573383877422));
#80477=CARTESIAN_POINT('Ctrl Pts',(16.9281666793966,-17.8471486364691,-17.3569535347569));
#80478=CARTESIAN_POINT('Ctrl Pts',(16.9204737498509,-17.8598088030428,-17.3560708139716));
#80479=CARTESIAN_POINT('Ctrl Pts',(16.9161692543657,-17.8669882701148,-17.3555735847864));
#80480=CARTESIAN_POINT('Ctrl Pts',(16.904778877573,-17.886244337519,-17.3542487688532));
#80481=CARTESIAN_POINT('Ctrl Pts',(16.8977699574249,-17.8983661491638,-17.3534239746956));
#80482=CARTESIAN_POINT('Ctrl Pts',(16.841012124919,-17.9988146452115,-17.3466623653921));
#80483=CARTESIAN_POINT('Ctrl Pts',(16.797542816139,-18.090546111532,-17.3409591144045));
#80484=CARTESIAN_POINT('Ctrl Pts',(16.7062965953606,-18.3253020389762,-17.327088482644));
#80485=CARTESIAN_POINT('Ctrl Pts',(16.66689522666,-18.4709554092311,-17.3191198229837));
#80486=CARTESIAN_POINT('Ctrl Pts',(16.6370543890108,-18.6586173482729,-17.3084710818138));
#80487=CARTESIAN_POINT('Ctrl Pts',(16.6319381894214,-18.6978542678952,-17.3062221120722));
#80488=CARTESIAN_POINT('Ctrl Pts',(16.6263939790653,-18.752216547317,-17.3030474639199));
#80489=CARTESIAN_POINT('Ctrl Pts',(16.6250239190544,-18.7672395315892,-17.302163979958));
#80490=CARTESIAN_POINT('Ctrl Pts',(16.6229323250401,-18.7932443177377,-17.3006220405579));
#80491=CARTESIAN_POINT('Ctrl Pts',(16.6221356451372,-18.8042196565844,-17.2999673810642));
#80492=CARTESIAN_POINT('Ctrl Pts',(16.6211102618329,-18.8200544997707,-17.2990166266043));
#80493=CARTESIAN_POINT('Ctrl Pts',(16.6208126721322,-18.8249095717865,-17.2987242743752));
#80494=CARTESIAN_POINT('Ctrl Pts',(16.6203235173838,-18.8333671970458,-17.2982134544967));
#80495=CARTESIAN_POINT('Ctrl Pts',(16.6201244222717,-18.8369693221453,-17.2979954085226));
#80496=CARTESIAN_POINT('Ctrl Pts',(16.6197264097709,-18.8445206026431,-17.2975372654557));
#80497=CARTESIAN_POINT('Ctrl Pts',(16.6195293495792,-18.8484697961352,-17.297297070256));
#80498=CARTESIAN_POINT('Ctrl Pts',(16.6190357980362,-18.8589506819446,-17.2966580745959));
#80499=CARTESIAN_POINT('Ctrl Pts',(16.6187585037423,-18.865483174457,-17.2962582227246));
#80500=CARTESIAN_POINT('Ctrl Pts',(16.6177066689221,-18.8933033043853,-17.2945489332139));
#80501=CARTESIAN_POINT('Ctrl Pts',(16.6172232249897,-18.9145998706016,-17.2932244419876));
#80502=CARTESIAN_POINT('Ctrl Pts',(16.6170218768584,-18.9410730857242,-17.29156108135));
#80503=CARTESIAN_POINT('Ctrl Pts',(16.6170014935722,-18.9462471117899,-17.2912351841013));
#80504=CARTESIAN_POINT('Ctrl Pts',(16.6169868170195,-18.9999278656385,-17.2878459960333));
#80505=CARTESIAN_POINT('Ctrl Pts',(16.6186407107698,-19.048417613827,-17.2847171524678));
#80506=CARTESIAN_POINT('Ctrl Pts',(16.6353861375546,-19.2926578549782,-17.2687464387349));
#80507=CARTESIAN_POINT('Ctrl Pts',(16.6759975329941,-19.4857400604894,-17.2555537953033));
#80508=CARTESIAN_POINT('Ctrl Pts',(16.7435636736328,-19.6730128904649,-17.2430395163305));
#80509=CARTESIAN_POINT('Ctrl Pts',(16.7444891185652,-19.6755625818381,-17.2428691667365));
#80510=CARTESIAN_POINT('Ctrl Pts',(16.7454194498739,-19.6781104569281,-17.2426989690604));
#80511=CARTESIAN_POINT('Origin',(18.734,-18.952,0.));
#80512=CARTESIAN_POINT('',(16.7454194329591,-19.6781104106039,-16.4437313840672));
#80513=CARTESIAN_POINT('',(16.7454194499739,-19.6781104572019,-16.6645989847956));
#80514=CARTESIAN_POINT('',(16.7454194499637,-19.6781104571739,0.));
#80515=CARTESIAN_POINT('',(16.6170007987637,-18.9530960249984,-16.7126929437736));
#80516=CARTESIAN_POINT('Ctrl Pts',(16.7454194499739,-19.6781104572019,-16.6645989847956));
#80517=CARTESIAN_POINT('Ctrl Pts',(16.7447285794631,-19.6762183874118,-16.6647267402562));
#80518=CARTESIAN_POINT('Ctrl Pts',(16.7440404071567,-19.6743253256948,-16.6648546065633));
#80519=CARTESIAN_POINT('Ctrl Pts',(16.6879393952875,-19.5193109532753,-16.675328438261));
#80520=CARTESIAN_POINT('Ctrl Pts',(16.6503766399063,-19.3603127697113,-16.6862947944489));
#80521=CARTESIAN_POINT('Ctrl Pts',(16.6218547097861,-19.1171078230942,-16.7022899066289));
#80522=CARTESIAN_POINT('Ctrl Pts',(16.6170428510306,-19.0351423589209,-16.7075611653873));
#80523=CARTESIAN_POINT('Ctrl Pts',(16.6170002849213,-18.9530983426379,-16.7126936923974));
#80524=CARTESIAN_POINT('Ctrl Pts',(16.6170002837491,-18.9530960809383,-16.7126938338853));
#80525=CARTESIAN_POINT('Ctrl Pts',(16.6169868619618,-18.9271728859926,-16.7143155418154));
#80526=CARTESIAN_POINT('Ctrl Pts',(16.6174495936263,-18.9012505641371,-16.715923233117));
#80527=CARTESIAN_POINT('Ctrl Pts',(16.6190263314276,-18.8577355919444,-16.718599006575));
#80528=CARTESIAN_POINT('Ctrl Pts',(16.6198840706988,-18.8401372970935,-16.7196748223783));
#80529=CARTESIAN_POINT('Ctrl Pts',(16.6214584275455,-18.8144384867155,-16.7212369178697));
#80530=CARTESIAN_POINT('Ctrl Pts',(16.6220021597015,-18.8063284834004,-16.721728583908));
#80531=CARTESIAN_POINT('Ctrl Pts',(16.6230473347477,-18.7919780147991,-16.7225963283517));
#80532=CARTESIAN_POINT('Ctrl Pts',(16.6235297739623,-18.7857363028034,-16.7229729989713));
#80533=CARTESIAN_POINT('Ctrl Pts',(16.6245388663628,-18.7733936660693,-16.7237163836535));
#80534=CARTESIAN_POINT('Ctrl Pts',(16.6250643172567,-18.7672927069112,-16.7240831317392));
#80535=CARTESIAN_POINT('Ctrl Pts',(16.626163866657,-18.7551428118738,-16.7248121241648));
#80536=CARTESIAN_POINT('Ctrl Pts',(16.6267375501404,-18.7490938982214,-16.725174377874));
#80537=CARTESIAN_POINT('Ctrl Pts',(16.6281714412872,-18.7346373835589,-16.7260385542006));
#80538=CARTESIAN_POINT('Ctrl Pts',(16.629055973347,-18.7262322575702,-16.7265397080837));
#80539=CARTESIAN_POINT('Ctrl Pts',(16.631901147117,-18.7006681922977,-16.7280602026543));
#80540=CARTESIAN_POINT('Ctrl Pts',(16.6340214765645,-18.6835274836393,-16.729074529535));
#80541=CARTESIAN_POINT('Ctrl Pts',(16.6419661876515,-18.6251729868462,-16.7325118371407));
#80542=CARTESIAN_POINT('Ctrl Pts',(16.6487962645608,-18.5841045300971,-16.734903572597));
#80543=CARTESIAN_POINT('Ctrl Pts',(16.6900265319096,-18.3745762578523,-16.7470133625295));
#80544=CARTESIAN_POINT('Ctrl Pts',(16.7436413674956,-18.2105702553108,-16.7561209259851));
#80545=CARTESIAN_POINT('Ctrl Pts',(16.8430671589661,-17.9980646740256,-16.7690150810144));
#80546=CARTESIAN_POINT('Ctrl Pts',(16.8721436967597,-17.9424904293108,-16.7725069238828));
#80547=CARTESIAN_POINT('Ctrl Pts',(16.9191779886948,-17.8615568448669,-16.777891277069));
#80548=CARTESIAN_POINT('Ctrl Pts',(16.935298360219,-17.8351663546488,-16.7796970804036));
#80549=CARTESIAN_POINT('Ctrl Pts',(16.955838015889,-17.8031397960092,-16.7819630062873));
#80550=CARTESIAN_POINT('Ctrl Pts',(16.9597163394809,-17.7971591889894,-16.782389404854));
#80551=CARTESIAN_POINT('Ctrl Pts',(16.9658647092424,-17.7877821157767,-16.7830632979736));
#80552=CARTESIAN_POINT('Ctrl Pts',(16.9681145509226,-17.7843723759453,-16.7833094605694));
#80553=CARTESIAN_POINT('Ctrl Pts',(16.9723521715762,-17.7779903260258,-16.7837723491849));
#80554=CARTESIAN_POINT('Ctrl Pts',(16.9743376166485,-17.7750165328631,-16.7839889190161));
#80555=CARTESIAN_POINT('Ctrl Pts',(16.978905371182,-17.7682123568627,-16.7844864535024));
#80556=CARTESIAN_POINT('Ctrl Pts',(16.9814926831268,-17.7643853977311,-16.784767753039));
#80557=CARTESIAN_POINT('Ctrl Pts',(16.9895487940191,-17.7525530505832,-16.7856419578467));
#80558=CARTESIAN_POINT('Ctrl Pts',(16.9950599851321,-17.7445768715979,-16.7862376289525));
#80559=CARTESIAN_POINT('Ctrl Pts',(17.05732849338,-17.6557681672781,-16.7929390074858));
#80560=CARTESIAN_POINT('Ctrl Pts',(17.1196150424624,-17.5789738219457,-16.7993722687496));
#80561=CARTESIAN_POINT('Ctrl Pts',(17.3015406410054,-17.3842341960491,-16.8169267170906));
#80562=CARTESIAN_POINT('Ctrl Pts',(17.4302425940965,-17.2756758752608,-16.8280724208305));
#80563=CARTESIAN_POINT('Ctrl Pts',(17.5967906324138,-17.1660996689677,-16.8405985752254));
#80564=CARTESIAN_POINT('Ctrl Pts',(17.6235430655295,-17.1493434326143,-16.8425611955875));
#80565=CARTESIAN_POINT('Ctrl Pts',(17.6638282754041,-17.1253483213788,-16.8454447197155));
#80566=CARTESIAN_POINT('Ctrl Pts',(17.6770802494969,-17.117648742606,-16.8463820279014));
#80567=CARTESIAN_POINT('Ctrl Pts',(17.7013526733181,-17.1038965027822,-16.8480787278338));
#80568=CARTESIAN_POINT('Ctrl Pts',(17.7123455632341,-17.0977968665062,-16.8488397815537));
#80569=CARTESIAN_POINT('Ctrl Pts',(17.7297375505029,-17.088348187627,-16.8500324660596));
#80570=CARTESIAN_POINT('Ctrl Pts',(17.7361004338387,-17.0849334229608,-16.8504664370605));
#80571=CARTESIAN_POINT('Ctrl Pts',(17.7425268570161,-17.0815267953092,-16.8509023811204));
#80572=CARTESIAN_POINT('Ctrl Pts',(17.7425729891198,-17.0815023430055,-16.8509055104243));
#80573=CARTESIAN_POINT('Ctrl Pts',(17.7426668794635,-17.0814525809145,-16.8509118790902));
#80574=CARTESIAN_POINT('Ctrl Pts',(17.7427146386244,-17.0814272707957,-16.8509151185059));
#80575=CARTESIAN_POINT('Ctrl Pts',(17.7428118423549,-17.0813757621387,-16.8509217113889));
#80576=CARTESIAN_POINT('Ctrl Pts',(17.7428612879522,-17.081349563224,-16.8509250649166));
#80577=CARTESIAN_POINT('Ctrl Pts',(17.7429619260082,-17.0812962449244,-16.8509318901631));
#80578=CARTESIAN_POINT('Ctrl Pts',(17.7430131194289,-17.0812691252103,-16.8509353619371));
#80579=CARTESIAN_POINT('Ctrl Pts',(17.7431173170041,-17.0812139320234,-16.8509424279772));
#80580=CARTESIAN_POINT('Ctrl Pts',(17.7431703219175,-17.081185858342,-16.850946022284));
#80581=CARTESIAN_POINT('Ctrl Pts',(17.7432782085371,-17.0811287228202,-16.8509533378366));
#80582=CARTESIAN_POINT('Ctrl Pts',(17.7433330911034,-17.081099660732,-16.8509570591291));
#80583=CARTESIAN_POINT('Ctrl Pts',(17.7434448015627,-17.0810405127361,-16.8509646332646));
#80584=CARTESIAN_POINT('Ctrl Pts',(17.7435016301821,-17.0810104266667,-16.8509684861445));
#80585=CARTESIAN_POINT('Ctrl Pts',(17.7436173038241,-17.0809491937557,-16.850976328236));
#80586=CARTESIAN_POINT('Ctrl Pts',(17.7436761494837,-17.080918046816,-16.8509803174775));
#80587=CARTESIAN_POINT('Ctrl Pts',(17.7437959307841,-17.0808546539457,-16.8509884372397));
#80588=CARTESIAN_POINT('Ctrl Pts',(17.7438568670515,-17.08082240794,-16.8509925677885));
#80589=CARTESIAN_POINT('Ctrl Pts',(17.7439809057941,-17.0807567773794,-16.851000975289));
#80590=CARTESIAN_POINT('Ctrl Pts',(17.7440440088359,-17.0807233927999,-16.8510052522637));
#80591=CARTESIAN_POINT('Ctrl Pts',(17.744172460018,-17.0806554441905,-16.8510139579162));
#80592=CARTESIAN_POINT('Ctrl Pts',(17.7442378087646,-17.0806208801353,-16.8510183866186));
#80593=CARTESIAN_POINT('Ctrl Pts',(17.7443708352629,-17.0805505290919,-16.851027401363));
#80594=CARTESIAN_POINT('Ctrl Pts',(17.7444385102685,-17.0805147438732,-16.8510319872011));
#80595=CARTESIAN_POINT('Ctrl Pts',(17.7445651192025,-17.0804478043335,-16.8510405660683));
#80596=CARTESIAN_POINT('Ctrl Pts',(17.7446240540237,-17.0804166484052,-16.8510445592212));
#80597=CARTESIAN_POINT('Ctrl Pts',(17.7447516746761,-17.0803491893842,-16.8510532057803));
#80598=CARTESIAN_POINT('Ctrl Pts',(17.7448203621204,-17.0803128867143,-16.8510578592246));
#80599=CARTESIAN_POINT('Ctrl Pts',(17.7449690843897,-17.0802342945335,-16.8510679342921));
#80600=CARTESIAN_POINT('Ctrl Pts',(17.7450491209302,-17.0801920058454,-16.8510733559352));
#80601=CARTESIAN_POINT('Ctrl Pts',(17.7452223913948,-17.0801004696195,-16.8510850924134));
#80602=CARTESIAN_POINT('Ctrl Pts',(17.7453156269186,-17.0800512235794,-16.8510914072264));
#80603=CARTESIAN_POINT('Ctrl Pts',(17.7455174354136,-17.079944649701,-16.8511050745769));
#80604=CARTESIAN_POINT('Ctrl Pts',(17.7456260101929,-17.0798873240781,-16.8511124270602));
#80605=CARTESIAN_POINT('Ctrl Pts',(17.7458609678064,-17.0797632966216,-16.8511283364974));
#80606=CARTESIAN_POINT('Ctrl Pts',(17.7459873521322,-17.0796965982846,-16.8511368933133));
#80607=CARTESIAN_POINT('Ctrl Pts',(17.7462732758041,-17.0795457413211,-16.8511562496328));
#80608=CARTESIAN_POINT('Ctrl Pts',(17.7464328191866,-17.0794615902696,-16.8511670488684));
#80609=CARTESIAN_POINT('Ctrl Pts',(17.7523042775245,-17.076365652558,-16.8515644249942));
#80610=CARTESIAN_POINT('Ctrl Pts',(17.7580299798871,-17.0733799697391,-16.851950074291));
#80611=CARTESIAN_POINT('Ctrl Pts',(17.7712868268408,-17.0665441172548,-16.8528387314697));
#80612=CARTESIAN_POINT('Ctrl Pts',(17.7788275960508,-17.062712774231,-16.8533410721469));
#80613=CARTESIAN_POINT('Ctrl Pts',(17.7991801830064,-17.052524954163,-16.8546885868926));
#80614=CARTESIAN_POINT('Ctrl Pts',(17.8120339262939,-17.0462528725238,-16.8555308132934));
#80615=CARTESIAN_POINT('Ctrl Pts',(17.9304939887427,-16.989928428021,-16.8632149915667));
#80616=CARTESIAN_POINT('Ctrl Pts',(18.0400179132035,-16.9485677221105,-16.8697401034514));
#80617=CARTESIAN_POINT('Ctrl Pts',(18.3090801895793,-16.8716919252939,-16.8850589580981));
#80618=CARTESIAN_POINT('Ctrl Pts',(18.4703755118528,-16.8451709323919,-16.8936690031478));
#80619=CARTESIAN_POINT('Ctrl Pts',(18.6653344442067,-16.8358677130347,-16.9048788398518));
#80620=CARTESIAN_POINT('Ctrl Pts',(18.6976039157534,-16.8350668684478,-16.9067617345747));
#80621=CARTESIAN_POINT('Ctrl Pts',(18.7371007728534,-16.8349899462351,-16.9091135022835));
#80622=CARTESIAN_POINT('Ctrl Pts',(18.7443244133671,-16.8350128518101,-16.9095455516763));
#80623=CARTESIAN_POINT('Ctrl Pts',(18.7556537446253,-16.8351067631316,-16.9102263895025));
#80624=CARTESIAN_POINT('Ctrl Pts',(18.7597596651064,-16.8351527452482,-16.9104737998769));
#80625=CARTESIAN_POINT('Ctrl Pts',(18.7674374807421,-16.8352610701164,-16.9109377275042));
#80626=CARTESIAN_POINT('Ctrl Pts',(18.7710093606906,-16.8353205086823,-16.9111540806862));
#80627=CARTESIAN_POINT('Ctrl Pts',(18.7791670149684,-16.8354769126114,-16.911649388466));
#80628=CARTESIAN_POINT('Ctrl Pts',(18.7837526198016,-16.8355797405529,-16.9119286667462));
#80629=CARTESIAN_POINT('Ctrl Pts',(18.7978618606407,-16.8359420068896,-16.9127905191966));
#80630=CARTESIAN_POINT('Ctrl Pts',(18.807383954816,-16.8362508289425,-16.9133757499156));
#80631=CARTESIAN_POINT('Ctrl Pts',(18.9364216048654,-16.8413079269359,-16.9213520338047));
#80632=CARTESIAN_POINT('Ctrl Pts',(19.0553143784831,-16.8561121280792,-16.9292199952126));
#80633=CARTESIAN_POINT('Ctrl Pts',(19.2789140605583,-16.9034317053216,-16.9443187785163));
#80634=CARTESIAN_POINT('Ctrl Pts',(19.3836298788765,-16.9341923064276,-16.951521706623));
#80635=CARTESIAN_POINT('Ctrl Pts',(19.5556677213986,-16.9995190604651,-16.9633455044071));
#80636=CARTESIAN_POINT('Ctrl Pts',(19.6243581520663,-17.0298698870102,-16.9680665544473));
#80637=CARTESIAN_POINT('Ctrl Pts',(19.7080738059936,-17.072313066918,-16.9738164718044));
#80638=CARTESIAN_POINT('Ctrl Pts',(19.7247354535037,-17.0810414106852,-16.9749608382613));
#80639=CARTESIAN_POINT('Ctrl Pts',(19.7488030543216,-17.0940611045734,-16.9766142763129));
#80640=CARTESIAN_POINT('Ctrl Pts',(19.7563024514415,-17.0981769557664,-16.9771295437616));
#80641=CARTESIAN_POINT('Ctrl Pts',(19.7694115851867,-17.1054753070374,-16.9780304179974));
#80642=CARTESIAN_POINT('Ctrl Pts',(19.7750320715254,-17.1086381744371,-16.9784167207105));
#80643=CARTESIAN_POINT('Ctrl Pts',(19.7859208829156,-17.1148314196666,-16.9791652681094));
#80644=CARTESIAN_POINT('Ctrl Pts',(19.7911907786622,-17.117858894421,-16.9795276123247));
#80645=CARTESIAN_POINT('Ctrl Pts',(19.8037626957109,-17.1251534546107,-16.9803922263226));
#80646=CARTESIAN_POINT('Ctrl Pts',(19.81105236395,-17.1294417062823,-16.9808937255789));
#80647=CARTESIAN_POINT('Ctrl Pts',(19.8372940336706,-17.1450911698053,-16.9826998226498));
#80648=CARTESIAN_POINT('Ctrl Pts',(19.8560939917438,-17.1567054912149,-16.9839951962583));
#80649=CARTESIAN_POINT('Ctrl Pts',(20.0311368845103,-17.2686682715246,-16.9960802779257));
#80650=CARTESIAN_POINT('Ctrl Pts',(20.1737172751414,-17.3888653358452,-17.0060122550063));
#80651=CARTESIAN_POINT('Ctrl Pts',(20.3527290484362,-17.5853189324434,-17.0205013874553));
#80652=CARTESIAN_POINT('Ctrl Pts',(20.4032560404005,-17.647514223404,-17.0249051360636));
#80653=CARTESIAN_POINT('Ctrl Pts',(20.4712215009817,-17.7416086132237,-17.0315447780943));
#80654=CARTESIAN_POINT('Ctrl Pts',(20.4915580853202,-17.771332781315,-17.0336394819498));
#80655=CARTESIAN_POINT('Ctrl Pts',(20.5151821465616,-17.8078256736547,-17.0362265599653));
#80656=CARTESIAN_POINT('Ctrl Pts',(20.5192056819206,-17.8141136270391,-17.0366728687045));
#80657=CARTESIAN_POINT('Ctrl Pts',(20.5254189178358,-17.8239376972936,-17.0373712172081));
#80658=CARTESIAN_POINT('Ctrl Pts',(20.5276316423008,-17.8274592808524,-17.0376217595799));
#80659=CARTESIAN_POINT('Ctrl Pts',(20.5317222171217,-17.8340122782707,-17.0380884032046));
#80660=CARTESIAN_POINT('Ctrl Pts',(20.5336027909015,-17.8370419244456,-17.0383043209604));
#80661=CARTESIAN_POINT('Ctrl Pts',(20.5378449737054,-17.8439148684098,-17.0387945329832));
#80662=CARTESIAN_POINT('Ctrl Pts',(20.5402019468074,-17.8477609522881,-17.0390691248937));
#80663=CARTESIAN_POINT('Ctrl Pts',(20.5462563197446,-17.8577116609078,-17.0397801942039));
#80664=CARTESIAN_POINT('Ctrl Pts',(20.5499351383302,-17.8638274458553,-17.0402178389317));
#80665=CARTESIAN_POINT('Ctrl Pts',(20.5723468941321,-17.9015156168502,-17.0429180080681));
#80666=CARTESIAN_POINT('Ctrl Pts',(20.5902856621675,-17.9335502427578,-17.0452268350105));
#80667=CARTESIAN_POINT('Ctrl Pts',(20.6867170429272,-18.1167741044773,-17.0584408359818));
#80668=CARTESIAN_POINT('Ctrl Pts',(20.7475690815485,-18.2765381088593,-17.0699344866839));
#80669=CARTESIAN_POINT('Ctrl Pts',(20.8116284131515,-18.5345466485141,-17.0872115149507));
#80670=CARTESIAN_POINT('Ctrl Pts',(20.8283439679135,-18.6286816855436,-17.0932786896403));
#80671=CARTESIAN_POINT('Ctrl Pts',(20.8409558102816,-18.7449146453183,-17.1004603605687));
#80672=CARTESIAN_POINT('Ctrl Pts',(20.8429419120807,-18.7662281106361,-17.1017650263321));
#80673=CARTESIAN_POINT('Ctrl Pts',(20.8453044658029,-18.796553331079,-17.1036045772717));
#80674=CARTESIAN_POINT('Ctrl Pts',(20.845947066957,-18.8055424822839,-17.1041477817932));
#80675=CARTESIAN_POINT('Ctrl Pts',(20.8469560595829,-18.8210485263731,-17.1050812784005));
#80676=CARTESIAN_POINT('Ctrl Pts',(20.8473497456271,-18.8275634607029,-17.105472422119));
#80677=CARTESIAN_POINT('Ctrl Pts',(20.8480455177565,-18.8400351780281,-17.1062191902275));
#80678=CARTESIAN_POINT('Ctrl Pts',(20.8483525711413,-18.8459916110184,-17.1065749668025));
#80679=CARTESIAN_POINT('Ctrl Pts',(20.8490849458517,-18.8614708124556,-17.1074973016845));
#80680=CARTESIAN_POINT('Ctrl Pts',(20.8494711332539,-18.8709953652404,-17.1080626293174));
#80681=CARTESIAN_POINT('Ctrl Pts',(20.8505663739781,-18.9034153135123,-17.1099796816219));
#80682=CARTESIAN_POINT('Ctrl Pts',(20.8509681820027,-18.9263199714303,-17.1113217975202));
#80683=CARTESIAN_POINT('Ctrl Pts',(20.8512294930595,-19.1258362738193,-17.1229163774947));
#80684=CARTESIAN_POINT('Ctrl Pts',(20.8293620217039,-19.3017776712722,-17.1324066359812));
#80685=CARTESIAN_POINT('Ctrl Pts',(20.7646786984319,-19.5565379749944,-17.1467108196941));
#80686=CARTESIAN_POINT('Ctrl Pts',(20.7383784614357,-19.638721758431,-17.151433132377));
#80687=CARTESIAN_POINT('Ctrl Pts',(20.6935122054658,-19.7541324046316,-17.1585043066941));
#80688=CARTESIAN_POINT('Ctrl Pts',(20.6789486538994,-19.7888266357435,-17.1606900429626));
#80689=CARTESIAN_POINT('Ctrl Pts',(20.6603586880015,-19.8300024841953,-17.1633780704574));
#80690=CARTESIAN_POINT('Ctrl Pts',(20.6572109370662,-19.8368761748025,-17.1638299946993));
#80691=CARTESIAN_POINT('Ctrl Pts',(20.6522658643476,-19.8475236145485,-17.1645352329974));
#80692=CARTESIAN_POINT('Ctrl Pts',(20.6504940333148,-19.8513092294148,-17.1647870014815));
#80693=CARTESIAN_POINT('Ctrl Pts',(20.6471906570234,-19.8583129768261,-17.1652547463598));
#80694=CARTESIAN_POINT('Ctrl Pts',(20.6456621918922,-19.8615324983697,-17.1654705317739));
#80695=CARTESIAN_POINT('Ctrl Pts',(20.6421925962735,-19.8687933878563,-17.1659589220415));
#80696=CARTESIAN_POINT('Ctrl Pts',(20.6402467642362,-19.872832435068,-17.1662318150648));
#80697=CARTESIAN_POINT('Ctrl Pts',(20.6344782275707,-19.8847097936444,-17.1670378067765));
#80698=CARTESIAN_POINT('Ctrl Pts',(20.6306199561418,-19.8925305888619,-17.1675730425713));
#80699=CARTESIAN_POINT('Ctrl Pts',(20.6028094446167,-19.9480360450982,-17.1714027852549));
#80700=CARTESIAN_POINT('Ctrl Pts',(20.5771120906545,-19.9948198922747,-17.1747944177196));
#80701=CARTESIAN_POINT('Ctrl Pts',(20.5406295266286,-20.0556704152153,-17.1793798390697));
#80702=CARTESIAN_POINT('Ctrl Pts',(20.5313936963559,-20.0706485185349,-17.18052311187));
#80703=CARTESIAN_POINT('Ctrl Pts',(20.4960022688965,-20.1264741635916,-17.1848351015557));
#80704=CARTESIAN_POINT('Ctrl Pts',(20.4686326062794,-20.1665332600283,-17.1880325757327));
#80705=CARTESIAN_POINT('Ctrl Pts',(20.3751393206793,-20.2937582976294,-17.1984619202417));
#80706=CARTESIAN_POINT('Ctrl Pts',(20.3036275260464,-20.3767548892263,-17.2056947196037));
#80707=CARTESIAN_POINT('Ctrl Pts',(20.1869267148664,-20.4926911218813,-17.2162683684722));
#80708=CARTESIAN_POINT('Ctrl Pts',(20.1463326182621,-20.5299868720245,-17.2197575951288));
#80709=CARTESIAN_POINT('Ctrl Pts',(20.0781788416052,-20.587863377476,-17.2253152909978));
#80710=CARTESIAN_POINT('Ctrl Pts',(20.0514942467233,-20.6094302018997,-17.2274222011303));
#80711=CARTESIAN_POINT('Ctrl Pts',(20.0157271166172,-20.6369277202113,-17.2301587782194));
#80712=CARTESIAN_POINT('Ctrl Pts',(20.0071077758976,-20.6434497987061,-17.2308117875296));
#80713=CARTESIAN_POINT('Ctrl Pts',(19.9929062851411,-20.6540257189612,-17.2318772931054));
#80714=CARTESIAN_POINT('Ctrl Pts',(19.9873536799611,-20.6581187348637,-17.2322913188467));
#80715=CARTESIAN_POINT('Ctrl Pts',(19.9765651495648,-20.6659902387322,-17.2330908347344));
#80716=CARTESIAN_POINT('Ctrl Pts',(19.9713317550894,-20.6697720508424,-17.2334764512315));
#80717=CARTESIAN_POINT('Ctrl Pts',(19.9592058797045,-20.6784504141309,-17.2343648686458));
#80718=CARTESIAN_POINT('Ctrl Pts',(19.9523011746944,-20.6833297580232,-17.2348670035122));
#80719=CARTESIAN_POINT('Ctrl Pts',(19.9336483210147,-20.6963443178347,-17.2362136017454));
#80720=CARTESIAN_POINT('Ctrl Pts',(19.9218466006839,-20.704402254458,-17.2370551237865));
#80721=CARTESIAN_POINT('Ctrl Pts',(19.8128220352967,-20.777234176032,-17.244736211265));
#80722=CARTESIAN_POINT('Ctrl Pts',(19.7104695089811,-20.8339801649476,-17.2512591668123));
#80723=CARTESIAN_POINT('Ctrl Pts',(19.4555753743655,-20.9488735719642,-17.266565339726));
#80724=CARTESIAN_POINT('Ctrl Pts',(19.3000076244706,-20.998411150779,-17.2751654658189));
#80725=CARTESIAN_POINT('Ctrl Pts',(19.1084209255003,-21.0358797194721,-17.2863744842733));
#80726=CARTESIAN_POINT('Ctrl Pts',(19.0763806304814,-21.0413829130412,-17.2882704544787));
#80727=CARTESIAN_POINT('Ctrl Pts',(19.037067009099,-21.0472068630164,-17.2906367699506));
#80728=CARTESIAN_POINT('Ctrl Pts',(19.0299003533086,-21.0482309959315,-17.2910697519764));
#80729=CARTESIAN_POINT('Ctrl Pts',(19.0186574245896,-21.0497788348875,-17.2917517357108));
#80730=CARTESIAN_POINT('Ctrl Pts',(19.0145845617733,-21.0503274750406,-17.2919993516869));
#80731=CARTESIAN_POINT('Ctrl Pts',(19.0069688193734,-21.0513307939579,-17.2924634529984));
#80732=CARTESIAN_POINT('Ctrl Pts',(19.0034263778175,-21.0517883667384,-17.2926797729726));
#80733=CARTESIAN_POINT('Ctrl Pts',(18.9953375389615,-21.0528123860249,-17.2931747252015));
#80734=CARTESIAN_POINT('Ctrl Pts',(18.9907904661317,-21.0533730383105,-17.2934536793413));
#80735=CARTESIAN_POINT('Ctrl Pts',(18.9768089142779,-21.0550509002867,-17.294313560248));
#80736=CARTESIAN_POINT('Ctrl Pts',(18.9673688572317,-21.0561193470884,-17.2948971263252));
#80737=CARTESIAN_POINT('Ctrl Pts',(18.8825100990503,-21.0651457761149,-17.3001678465681));
#80738=CARTESIAN_POINT('Ctrl Pts',(18.806729387204,-21.0691084564982,-17.3050497269885));
#80739=CARTESIAN_POINT('Ctrl Pts',(18.5459858057495,-21.0687277182614,-17.3221026647377));
#80740=CARTESIAN_POINT('Ctrl Pts',(18.3618555908207,-21.0442270342742,-17.3344994882983));
#80741=CARTESIAN_POINT('Ctrl Pts',(18.1318214783832,-20.9822479470869,-17.3495264397384));
#80742=CARTESIAN_POINT('Ctrl Pts',(18.0809327593344,-20.9664551810059,-17.3528279669364));
#80743=CARTESIAN_POINT('Ctrl Pts',(18.018861844955,-20.9445922023598,-17.3568295848838));
#80744=CARTESIAN_POINT('Ctrl Pts',(18.0070706217971,-20.9403208884438,-17.3575886336221));
#80745=CARTESIAN_POINT('Ctrl Pts',(17.9884944316745,-20.9334044163272,-17.3587828592442));
#80746=CARTESIAN_POINT('Ctrl Pts',(17.9816841035877,-20.9308286453137,-17.3592203398635));
#80747=CARTESIAN_POINT('Ctrl Pts',(17.9689419835707,-20.9259340899503,-17.3600382710444));
#80748=CARTESIAN_POINT('Ctrl Pts',(17.9630071203189,-20.9236235799011,-17.3604189934957));
#80749=CARTESIAN_POINT('Ctrl Pts',(17.9497498742878,-20.9183933685983,-17.361268944669));
#80750=CARTESIAN_POINT('Ctrl Pts',(17.9424331662305,-20.9154594699138,-17.3617376895754));
#80751=CARTESIAN_POINT('Ctrl Pts',(17.9239378049553,-20.9079228976669,-17.3629218176192));
#80752=CARTESIAN_POINT('Ctrl Pts',(17.9127817811841,-20.9032651761447,-17.3636353351782));
#80753=CARTESIAN_POINT('Ctrl Pts',(17.8493602283988,-20.876145945981,-17.3676884274963));
#80754=CARTESIAN_POINT('Ctrl Pts',(17.7979742561163,-20.8516793899288,-17.3709588925312));
#80755=CARTESIAN_POINT('Ctrl Pts',(17.7238752779461,-20.8126606260659,-17.3756896508523));
#80756=CARTESIAN_POINT('Ctrl Pts',(17.7003574321009,-20.7996993886095,-17.3771935568014));
#80757=CARTESIAN_POINT('Ctrl Pts',(17.5767171564955,-20.7284586784432,-17.3851309162804));
#80758=CARTESIAN_POINT('Ctrl Pts',(17.481259293531,-20.6624825405355,-17.3913558095641));
#80759=CARTESIAN_POINT('Ctrl Pts',(17.3297857736773,-20.538277826611,-17.4020347080446));
#80760=CARTESIAN_POINT('Ctrl Pts',(17.2708273778643,-20.4840635801267,-17.4064365281268));
#80761=CARTESIAN_POINT('Ctrl Pts',(17.190006383073,-20.4008163593799,-17.4130735474593));
#80762=CARTESIAN_POINT('Ctrl Pts',(17.1655931027784,-20.374351781112,-17.4151676854633));
#80763=CARTESIAN_POINT('Ctrl Pts',(17.1369483247276,-20.3416656668973,-17.4177541356966));
#80764=CARTESIAN_POINT('Ctrl Pts',(17.1320583846019,-20.3360259305138,-17.4182004086209));
#80765=CARTESIAN_POINT('Ctrl Pts',(17.1244905989249,-20.3272039065964,-17.4188987131706));
#80766=CARTESIAN_POINT('Ctrl Pts',(17.1217920767779,-20.3240393246855,-17.4191492477084));
#80767=CARTESIAN_POINT('Ctrl Pts',(17.1167971590114,-20.3181466564993,-17.4196158843617));
#80768=CARTESIAN_POINT('Ctrl Pts',(17.1144983247872,-20.3154207125252,-17.4198318030281));
#80769=CARTESIAN_POINT('Ctrl Pts',(17.1093069350145,-20.3092331392292,-17.4203220269863));
#80770=CARTESIAN_POINT('Ctrl Pts',(17.1064185647059,-20.3057680821503,-17.420596629983));
#80771=CARTESIAN_POINT('Ctrl Pts',(17.0978965642405,-20.2954779001013,-17.4214122749751));
#80772=CARTESIAN_POINT('Ctrl Pts',(17.0922947139665,-20.2886267497324,-17.4219555296657));
#80773=CARTESIAN_POINT('Ctrl Pts',(17.05110318643,-20.2375992746436,-17.4260018982156));
#80774=CARTESIAN_POINT('Ctrl Pts',(17.0172621886901,-20.1920472768033,-17.4296147071732));
#80775=CARTESIAN_POINT('Ctrl Pts',(16.9504045590503,-20.0940631314751,-17.4372973967215));
#80776=CARTESIAN_POINT('Ctrl Pts',(16.9177756663548,-20.0414262112772,-17.4413750699095));
#80777=CARTESIAN_POINT('Ctrl Pts',(16.833894641212,-19.8918409600347,-17.4527032348205));
#80778=CARTESIAN_POINT('Ctrl Pts',(16.7877887117364,-19.7922181179369,-17.4599518152647));
#80779=CARTESIAN_POINT('Ctrl Pts',(16.7481977200789,-19.6856856149317,-17.4672585804267));
#80780=CARTESIAN_POINT('Ctrl Pts',(16.7468031555774,-19.6818999771293,-17.4675176808637));
#80781=CARTESIAN_POINT('Ctrl Pts',(16.745419450228,-19.6781104578977,-17.467776498566));
#80782=CARTESIAN_POINT('',(16.6170006442199,-18.9503484472246,-16.4878149124144));
#80783=CARTESIAN_POINT('Ctrl Pts',(16.7454194498739,-19.6781104569281,-17.2426989690604));
#80784=CARTESIAN_POINT('Ctrl Pts',(16.7608133381091,-19.720269313674,-17.2398827637156));
#80785=CARTESIAN_POINT('Ctrl Pts',(16.7775450772594,-19.761930911878,-17.2371085316352));
#80786=CARTESIAN_POINT('Ctrl Pts',(16.8006203767587,-19.8144898912909,-17.2336175673096));
#80787=CARTESIAN_POINT('Ctrl Pts',(16.8057522414893,-19.8259028392701,-17.2328600420512));
#80788=CARTESIAN_POINT('Ctrl Pts',(16.8140577700572,-19.8439444070767,-17.2316632137377));
#80789=CARTESIAN_POINT('Ctrl Pts',(16.817165214111,-19.8506030254568,-17.2312216439893));
#80790=CARTESIAN_POINT('Ctrl Pts',(16.8230280590925,-19.8629971052561,-17.2303999472867));
#80791=CARTESIAN_POINT('Ctrl Pts',(16.8257747635559,-19.8687365668966,-17.2300195250802));
#80792=CARTESIAN_POINT('Ctrl Pts',(16.8319433148699,-19.8814784057187,-17.2291751312795));
#80793=CARTESIAN_POINT('Ctrl Pts',(16.8353780490435,-19.8884744684066,-17.2287116140876));
#80794=CARTESIAN_POINT('Ctrl Pts',(16.8455036916702,-19.9088142507746,-17.2273642260543));
#80795=CARTESIAN_POINT('Ctrl Pts',(16.8522972775726,-19.9221065397874,-17.2264839527934));
#80796=CARTESIAN_POINT('Ctrl Pts',(16.9092402998089,-20.030671754689,-17.2192939161027));
#80797=CARTESIAN_POINT('Ctrl Pts',(16.9664531715157,-20.122069809812,-17.2132499545465));
#80798=CARTESIAN_POINT('Ctrl Pts',(17.109751978709,-20.3163257349589,-17.1999842959857));
#80799=CARTESIAN_POINT('Ctrl Pts',(17.1991351650164,-20.4161561880625,-17.1928656132533));
#80800=CARTESIAN_POINT('Ctrl Pts',(17.3093860429016,-20.5180247310711,-17.1845197435298));
#80801=CARTESIAN_POINT('Ctrl Pts',(17.3215698782723,-20.5290223577061,-17.1836024659585));
#80802=CARTESIAN_POINT('Ctrl Pts',(17.3736850652844,-20.5749752300406,-17.1796940207168));
#80803=CARTESIAN_POINT('Ctrl Pts',(17.4147922239866,-20.6085612447708,-17.1766482415168));
#80804=CARTESIAN_POINT('Ctrl Pts',(17.4640562984496,-20.6458145583144,-17.1729828814155));
#80805=CARTESIAN_POINT('Ctrl Pts',(17.4710311312166,-20.6510215989395,-17.1724635928918));
#80806=CARTESIAN_POINT('Ctrl Pts',(17.4816439613699,-20.6588431154939,-17.1716725967923));
#80807=CARTESIAN_POINT('Ctrl Pts',(17.4852585715187,-20.6614893718151,-17.1714030440656));
#80808=CARTESIAN_POINT('Ctrl Pts',(17.4917636998961,-20.666220136105,-17.1709176169094));
#80809=CARTESIAN_POINT('Ctrl Pts',(17.4946511041306,-20.6683088341939,-17.1707020374017));
#80810=CARTESIAN_POINT('Ctrl Pts',(17.5009388064773,-20.6728331082946,-17.1702323235958));
#80811=CARTESIAN_POINT('Ctrl Pts',(17.5043410081815,-20.6752658694224,-17.169978007079));
#80812=CARTESIAN_POINT('Ctrl Pts',(17.5139234868172,-20.6820750420492,-17.1692613151904));
#80813=CARTESIAN_POINT('Ctrl Pts',(17.5201199972535,-20.6864283450447,-17.1687974052941));
#80814=CARTESIAN_POINT('Ctrl Pts',(17.5574222943183,-20.7123369299239,-17.1660026228435));
#80815=CARTESIAN_POINT('Ctrl Pts',(17.5890761154363,-20.7330867728352,-17.1636224197635));
#80816=CARTESIAN_POINT('Ctrl Pts',(17.6953529688962,-20.7987499626778,-17.1556463562796));
#80817=CARTESIAN_POINT('Ctrl Pts',(17.7721887097019,-20.8399063014434,-17.149907405615));
#80818=CARTESIAN_POINT('Ctrl Pts',(18.0106979530405,-20.9493141414109,-17.1325699008923));
#80819=CARTESIAN_POINT('Ctrl Pts',(18.1785589325585,-21.0023507636008,-17.1210593388659));
#80820=CARTESIAN_POINT('Ctrl Pts',(18.3736831637739,-21.0382381905442,-17.1088475285528));
#80821=CARTESIAN_POINT('Ctrl Pts',(18.3963709338924,-21.0420298297795,-17.1074434360905));
#80822=CARTESIAN_POINT('Ctrl Pts',(18.4285581431009,-21.0468712202328,-17.1054730705881));
#80823=CARTESIAN_POINT('Ctrl Pts',(18.4380091888165,-21.0482274689719,-17.1048971398273));
#80824=CARTESIAN_POINT('Ctrl Pts',(18.4533813732738,-21.0503273796725,-17.1039645592587));
#80825=CARTESIAN_POINT('Ctrl Pts',(18.459296972004,-21.0511100146233,-17.1036066812973));
#80826=CARTESIAN_POINT('Ctrl Pts',(18.4716873170801,-21.0526959852523,-17.1028591653505));
#80827=CARTESIAN_POINT('Ctrl Pts',(18.4781626357032,-21.0534944231606,-17.1024696857292));
#80828=CARTESIAN_POINT('Ctrl Pts',(18.4935773304073,-21.0553228260666,-17.1015452736181));
#80829=CARTESIAN_POINT('Ctrl Pts',(18.502519832215,-21.0563257605315,-17.1010111984618));
#80830=CARTESIAN_POINT('Ctrl Pts',(18.5326744604026,-21.0595131652074,-17.0992174794108));
#80831=CARTESIAN_POINT('Ctrl Pts',(18.5539135556114,-21.0614341980435,-17.0979661196598));
#80832=CARTESIAN_POINT('Ctrl Pts',(18.6697334727688,-21.0701477840668,-17.0912024154926));
#80833=CARTESIAN_POINT('Ctrl Pts',(18.7646651557298,-21.0709013431714,-17.0858832799327));
#80834=CARTESIAN_POINT('Ctrl Pts',(19.028529215096,-21.0552518385551,-17.0713393476969));
#80835=CARTESIAN_POINT('Ctrl Pts',(19.1958840140949,-21.024936900985,-17.0624206444878));
#80836=CARTESIAN_POINT('Ctrl Pts',(19.3943175094104,-20.963747711953,-17.0505774117002));
#80837=CARTESIAN_POINT('Ctrl Pts',(19.4305054318287,-20.9515069006588,-17.0483610129389));
#80838=CARTESIAN_POINT('Ctrl Pts',(19.4731203919463,-20.9357949167947,-17.0456612832462));
#80839=CARTESIAN_POINT('Ctrl Pts',(19.4798879872012,-20.9332602890218,-17.0452298166369));
#80840=CARTESIAN_POINT('Ctrl Pts',(19.4908840459019,-20.9290776757838,-17.0445241115834));
#80841=CARTESIAN_POINT('Ctrl Pts',(19.4951204853496,-20.9274506323682,-17.0442510958433));
#80842=CARTESIAN_POINT('Ctrl Pts',(19.5026783434633,-20.9245200468903,-17.0437619570049));
#80843=CARTESIAN_POINT('Ctrl Pts',(19.5060017278716,-20.9232217183765,-17.0435461485296));
#80844=CARTESIAN_POINT('Ctrl Pts',(19.513173647039,-20.9203989845235,-17.0430788559055));
#80845=CARTESIAN_POINT('Ctrl Pts',(19.5170209436177,-20.9188717130743,-17.0428272053239));
#80846=CARTESIAN_POINT('Ctrl Pts',(19.5277103026619,-20.9145919967092,-17.042125347873));
#80847=CARTESIAN_POINT('Ctrl Pts',(19.5345424211642,-20.9118150979959,-17.0416737047906));
#80848=CARTESIAN_POINT('Ctrl Pts',(19.5733080544851,-20.8958223686678,-17.0390942672009));
#80849=CARTESIAN_POINT('Ctrl Pts',(19.604926719919,-20.881862622319,-17.0369254057522));
#80850=CARTESIAN_POINT('Ctrl Pts',(19.7038743504449,-20.8352501164384,-17.0299622041732));
#80851=CARTESIAN_POINT('Ctrl Pts',(19.7698188607241,-20.7998000452166,-17.0250595697919));
#80852=CARTESIAN_POINT('Ctrl Pts',(19.9994199025862,-20.6602140366031,-17.0073366904222));
#80853=CARTESIAN_POINT('Ctrl Pts',(20.1505147734033,-20.5371814167816,-16.9945245030053));
#80854=CARTESIAN_POINT('Ctrl Pts',(20.2971798395324,-20.3797973900105,-16.9813073144602));
#80855=CARTESIAN_POINT('Ctrl Pts',(20.3113709528804,-20.3641039358507,-16.9800173556114));
#80856=CARTESIAN_POINT('Ctrl Pts',(20.3308017985663,-20.3419575462654,-16.9782348656409));
#80857=CARTESIAN_POINT('Ctrl Pts',(20.3362420327966,-20.3356829245671,-16.9777339751764));
#80858=CARTESIAN_POINT('Ctrl Pts',(20.3455734683754,-20.3247914656884,-16.9768715754523));
#80859=CARTESIAN_POINT('Ctrl Pts',(20.3494820702649,-20.3201897288262,-16.9765093486441));
#80860=CARTESIAN_POINT('Ctrl Pts',(20.357539689041,-20.3106205380405,-16.9757605045732));
#80861=CARTESIAN_POINT('Ctrl Pts',(20.3616857239668,-20.3056506468461,-16.9753740118534));
#80862=CARTESIAN_POINT('Ctrl Pts',(20.3713500024069,-20.2939573845309,-16.9744702903082));
#80863=CARTESIAN_POINT('Ctrl Pts',(20.3768497578128,-20.2872188318682,-16.973953815822));
#80864=CARTESIAN_POINT('Ctrl Pts',(20.3946060463662,-20.2651872102885,-16.9722790123744));
#80865=CARTESIAN_POINT('Ctrl Pts',(20.406692005351,-20.249757521216,-16.9711275213006));
#80866=CARTESIAN_POINT('Ctrl Pts',(20.4676142374132,-20.1697151343637,-16.965259176585));
#80867=CARTESIAN_POINT('Ctrl Pts',(20.5129305547886,-20.1025027703689,-16.9606809236321));
#80868=CARTESIAN_POINT('Ctrl Pts',(20.6403754894141,-19.8878699686321,-16.946845481282));
#80869=CARTESIAN_POINT('Ctrl Pts',(20.7088263484278,-19.7331358983087,-16.9379734116954));
#80870=CARTESIAN_POINT('Ctrl Pts',(20.7740118195889,-19.5202936294107,-16.9254615545825));
#80871=CARTESIAN_POINT('Ctrl Pts',(20.7878439982756,-19.4680713616,-16.9223639644062));
#80872=CARTESIAN_POINT('Ctrl Pts',(20.8015776565788,-19.4068495453228,-16.9186407751822));
#80873=CARTESIAN_POINT('Ctrl Pts',(20.8034388880319,-19.3983050051234,-16.9181190839369));
#80874=CARTESIAN_POINT('Ctrl Pts',(20.8061752264278,-19.3853577945994,-16.9173251402454));
#80875=CARTESIAN_POINT('Ctrl Pts',(20.8070893834219,-19.3809633488445,-16.917055066754));
#80876=CARTESIAN_POINT('Ctrl Pts',(20.8087043779408,-19.3730741604594,-16.9165690857206));
#80877=CARTESIAN_POINT('Ctrl Pts',(20.809410370695,-19.3695805280093,-16.9163534760681));
#80878=CARTESIAN_POINT('Ctrl Pts',(20.8109243312331,-19.3619899506241,-16.9158841457757));
#80879=CARTESIAN_POINT('Ctrl Pts',(20.8117289904723,-19.3578924472523,-16.9156302453674));
#80880=CARTESIAN_POINT('Ctrl Pts',(20.8139529194793,-19.3463877955289,-16.9149158755395));
#80881=CARTESIAN_POINT('Ctrl Pts',(20.8153447206003,-19.3389754909675,-16.9144538871779));
#80882=CARTESIAN_POINT('Ctrl Pts',(20.8233854198353,-19.2948546302163,-16.9116943315946));
#80883=CARTESIAN_POINT('Ctrl Pts',(20.8291022163494,-19.2579853568534,-16.909348839196));
#80884=CARTESIAN_POINT('Ctrl Pts',(20.8446390631089,-19.1366973034976,-16.9015453574746));
#80885=CARTESIAN_POINT('Ctrl Pts',(20.850350781311,-19.0518391556437,-16.8959504851851));
#80886=CARTESIAN_POINT('Ctrl Pts',(20.8522009215649,-18.7885117643345,-16.8785545586206));
#80887=CARTESIAN_POINT('Ctrl Pts',(20.8309074044943,-18.6106680750795,-16.8668318577111));
#80888=CARTESIAN_POINT('Ctrl Pts',(20.7820171741914,-18.4154994476065,-16.8544504481824));
#80889=CARTESIAN_POINT('Ctrl Pts',(20.7761297522396,-18.3935079884013,-16.8530610021513));
#80890=CARTESIAN_POINT('Ctrl Pts',(20.767281718803,-18.3624706382347,-16.8511074365896));
#80891=CARTESIAN_POINT('Ctrl Pts',(20.764613238919,-18.3533437589543,-16.8505338812383));
#80892=CARTESIAN_POINT('Ctrl Pts',(20.7601722662553,-18.3385259014823,-16.8496040959525));
#80893=CARTESIAN_POINT('Ctrl Pts',(20.7584370954151,-18.332823958853,-16.8492466524165));
#80894=CARTESIAN_POINT('Ctrl Pts',(20.7547502605002,-18.3208898415695,-16.8484992092437));
#80895=CARTESIAN_POINT('Ctrl Pts',(20.752793789441,-18.3146592084495,-16.8481093716364));
#80896=CARTESIAN_POINT('Ctrl Pts',(20.7480626355886,-18.2998326237891,-16.8471825892301));
#80897=CARTESIAN_POINT('Ctrl Pts',(20.7452616936003,-18.2912451359431,-16.8466465136296));
#80898=CARTESIAN_POINT('Ctrl Pts',(20.735599876556,-18.2622534336926,-16.8448389090109));
#80899=CARTESIAN_POINT('Ctrl Pts',(20.7284826382223,-18.2419356031438,-16.843575842695));
#80900=CARTESIAN_POINT('Ctrl Pts',(20.6587625341826,-18.052228159565,-16.8318084486334));
#80901=CARTESIAN_POINT('Ctrl Pts',(20.5750396925942,-17.8913964400097,-16.8221122767492));
#80902=CARTESIAN_POINT('Ctrl Pts',(20.4037872425938,-17.6451980469061,-16.8057870189803));
#80903=CARTESIAN_POINT('Ctrl Pts',(20.3275183156282,-17.5532105615416,-16.7992370027396));
#80904=CARTESIAN_POINT('Ctrl Pts',(20.2372586948839,-17.4613649868366,-16.7916053244576));
#80905=CARTESIAN_POINT('Ctrl Pts',(20.2305472092367,-17.4546270040145,-16.7910384557641));
#80906=CARTESIAN_POINT('Ctrl Pts',(20.22053426422,-17.4447090892447,-16.7901932030767));
#80907=CARTESIAN_POINT('Ctrl Pts',(20.2172674023483,-17.4414941838675,-16.7899175001571));
#80908=CARTESIAN_POINT('Ctrl Pts',(20.2114360080532,-17.435792691584,-16.7894254381044));
#80909=CARTESIAN_POINT('Ctrl Pts',(20.2088755971124,-17.4333019612841,-16.7892094088383));
#80910=CARTESIAN_POINT('Ctrl Pts',(20.2033567500202,-17.4279604270036,-16.7887437993385));
#80911=CARTESIAN_POINT('Ctrl Pts',(20.2003963590415,-17.4251117930851,-16.7884940641518));
#80912=CARTESIAN_POINT('Ctrl Pts',(20.1922007241211,-17.4172713678801,-16.7878028062736));
#80913=CARTESIAN_POINT('Ctrl Pts',(20.1869482155621,-17.4122978192224,-16.7873599158284));
#80914=CARTESIAN_POINT('Ctrl Pts',(20.1580142745287,-17.3851804480279,-16.7849214477747));
#80915=CARTESIAN_POINT('Ctrl Pts',(20.133853401822,-17.3635572564836,-16.7828897892502));
#80916=CARTESIAN_POINT('Ctrl Pts',(19.98543406416,-17.2367432253775,-16.7704862553441));
#80917=CARTESIAN_POINT('Ctrl Pts',(19.8498790234841,-17.1456204884811,-16.7595226115642));
#80918=CARTESIAN_POINT('Ctrl Pts',(19.6013627714859,-17.0173079933107,-16.7412534803143));
#80919=CARTESIAN_POINT('Ctrl Pts',(19.4932278867572,-16.9723706974251,-16.7338079034804));
#80920=CARTESIAN_POINT('Ctrl Pts',(19.3683385792524,-16.9322210383114,-16.7257980479885));
#80921=CARTESIAN_POINT('Ctrl Pts',(19.3547141709729,-16.9279924849947,-16.724931577184));
#80922=CARTESIAN_POINT('Ctrl Pts',(19.3329551158053,-16.9214795917772,-16.7235591940653));
#80923=CARTESIAN_POINT('Ctrl Pts',(19.3248479202649,-16.9191057338591,-16.7230503664338));
#80924=CARTESIAN_POINT('Ctrl Pts',(19.3105204631249,-16.9150034782016,-16.7221554918337));
#80925=CARTESIAN_POINT('Ctrl Pts',(19.3043061381691,-16.9132548995965,-16.7217687910603));
#80926=CARTESIAN_POINT('Ctrl Pts',(19.2914323989594,-16.9096959717912,-16.7209706256762));
#80927=CARTESIAN_POINT('Ctrl Pts',(19.284771928854,-16.9078897027881,-16.7205592976642));
#80928=CARTESIAN_POINT('Ctrl Pts',(19.2676444147524,-16.9033346417586,-16.719505645151));
#80929=CARTESIAN_POINT('Ctrl Pts',(19.2571648286956,-16.900633460336,-16.7188648673748));
#80930=CARTESIAN_POINT('Ctrl Pts',(19.2132695484185,-16.8896774203105,-16.7161967173036));
#80931=CARTESIAN_POINT('Ctrl Pts',(19.1796746584067,-16.882157489057,-16.7141930430451));
#80932=CARTESIAN_POINT('Ctrl Pts',(19.0916091003971,-16.8646884938097,-16.7090282793365));
#80933=CARTESIAN_POINT('Ctrl Pts',(19.0369042807986,-16.8560507539028,-16.7059069956425));
#80934=CARTESIAN_POINT('Ctrl Pts',(18.8731176615586,-16.8367369042163,-16.6967386492996));
#80935=CARTESIAN_POINT('Ctrl Pts',(18.763479979485,-16.8323718538326,-16.6908402341054));
#80936=CARTESIAN_POINT('Ctrl Pts',(18.5938601737218,-16.8387864509178,-16.6815976616243));
#80937=CARTESIAN_POINT('Ctrl Pts',(18.5338497145011,-16.8436238732439,-16.6783024020314));
#80938=CARTESIAN_POINT('Ctrl Pts',(18.4161592016012,-16.8581809452183,-16.6716603173663));
#80939=CARTESIAN_POINT('Ctrl Pts',(18.3585155632465,-16.8677468619627,-16.6683205330776));
#80940=CARTESIAN_POINT('Ctrl Pts',(18.292624137677,-16.8815035010199,-16.6643275489039));
#80941=CARTESIAN_POINT('Ctrl Pts',(18.2839130739329,-16.8833796489422,-16.6637960873633));
#80942=CARTESIAN_POINT('Ctrl Pts',(18.2707977188182,-16.8862911352157,-16.6629901673629));
#80943=CARTESIAN_POINT('Ctrl Pts',(18.2663843508655,-16.8872857168237,-16.6627179871656));
#80944=CARTESIAN_POINT('Ctrl Pts',(18.2584971197321,-16.8890897416922,-16.6622297498418));
#80945=CARTESIAN_POINT('Ctrl Pts',(18.2550220843796,-16.8898938244951,-16.6620140025918));
#80946=CARTESIAN_POINT('Ctrl Pts',(18.2475087902232,-16.8916523301257,-16.6615461528995));
#80947=CARTESIAN_POINT('Ctrl Pts',(18.2434713563658,-16.8926098312757,-16.6612938803223));
#80948=CARTESIAN_POINT('Ctrl Pts',(18.2322211407829,-16.895312846393,-16.6605885706356));
#80949=CARTESIAN_POINT('Ctrl Pts',(18.2250147656582,-16.8970844059083,-16.6601340746958));
#80950=CARTESIAN_POINT('Ctrl Pts',(18.1835905623223,-16.9074990785256,-16.6575065042065));
#80951=CARTESIAN_POINT('Ctrl Pts',(18.1495859426044,-16.9169583693435,-16.655290583589));
#80952=CARTESIAN_POINT('Ctrl Pts',(18.0417718274778,-16.9498746348247,-16.6481093977352));
#80953=CARTESIAN_POINT('Ctrl Pts',(17.9690089488369,-16.9765322364171,-16.6430286910299));
#80954=CARTESIAN_POINT('Ctrl Pts',(17.727659407066,-17.0802906230617,-16.6256920557288));
#80955=CARTESIAN_POINT('Ctrl Pts',(17.567747693774,-17.1755147528589,-16.6134598082781));
#80956=CARTESIAN_POINT('Ctrl Pts',(17.4027686880646,-17.3057530074339,-16.6004987701282));
#80957=CARTESIAN_POINT('Ctrl Pts',(17.3835444186322,-17.3214860406576,-16.5989806449776));
#80958=CARTESIAN_POINT('Ctrl Pts',(17.357083333934,-17.3439307643588,-16.5968791102854));
#80959=CARTESIAN_POINT('Ctrl Pts',(17.3496103738568,-17.3503597344983,-16.5962842401266));
#80960=CARTESIAN_POINT('Ctrl Pts',(17.3376431755914,-17.3608014230724,-16.595329306469));
#80961=CARTESIAN_POINT('Ctrl Pts',(17.3331207510334,-17.3647814821929,-16.5949678968203));
#80962=CARTESIAN_POINT('Ctrl Pts',(17.3240615457209,-17.3728231155704,-16.5942428137148));
#80963=CARTESIAN_POINT('Ctrl Pts',(17.3195251758366,-17.3768850676299,-16.5938791611097));
#80964=CARTESIAN_POINT('Ctrl Pts',(17.3088168713055,-17.3865570553455,-16.5930193487606));
#80965=CARTESIAN_POINT('Ctrl Pts',(17.3026604104845,-17.3921841308002,-16.5925239142729));
#80966=CARTESIAN_POINT('Ctrl Pts',(17.2835121501476,-17.4098946901846,-16.5909793473806));
#80967=CARTESIAN_POINT('Ctrl Pts',(17.2706386846395,-17.4221054028918,-16.5899356515955));
#80968=CARTESIAN_POINT('Ctrl Pts',(17.2410243399071,-17.4509109877491,-16.5875210324327));
#80969=CARTESIAN_POINT('Ctrl Pts',(17.2244039201489,-17.4676266364197,-16.5861553944354));
#80970=CARTESIAN_POINT('Ctrl Pts',(17.1679676918297,-17.5263147711664,-16.5814760427944));
#80971=CARTESIAN_POINT('Ctrl Pts',(17.1295938981425,-17.5696406574505,-16.5782202756028));
#80972=CARTESIAN_POINT('Ctrl Pts',(16.9903283854136,-17.7405017733826,-16.5659901996405));
#80973=CARTESIAN_POINT('Ctrl Pts',(16.9024811696542,-17.877918134153,-16.5574141688273));
#80974=CARTESIAN_POINT('Ctrl Pts',(16.8041932721513,-18.0794530417435,-16.5448862244106));
#80975=CARTESIAN_POINT('Ctrl Pts',(16.7795980725527,-18.1360319846932,-16.5413681963752));
#80976=CARTESIAN_POINT('Ctrl Pts',(16.7542382247236,-18.202122879313,-16.5371698402641));
#80977=CARTESIAN_POINT('Ctrl Pts',(16.7510222061416,-18.2106691391418,-16.5366252730384));
#80978=CARTESIAN_POINT('Ctrl Pts',(16.7463011558343,-18.2234654228872,-16.5358070208537));
#80979=CARTESIAN_POINT('Ctrl Pts',(16.7447542002184,-18.2277000121953,-16.5355357742192));
#80980=CARTESIAN_POINT('Ctrl Pts',(16.7420079791541,-18.2352925957539,-16.5350485397713));
#80981=CARTESIAN_POINT('Ctrl Pts',(16.740803661073,-18.2386487060184,-16.5348328565262));
#80982=CARTESIAN_POINT('Ctrl Pts',(16.7382123271679,-18.2459278517811,-16.5343643644504));
#80983=CARTESIAN_POINT('Ctrl Pts',(16.7368284154959,-18.2498518853688,-16.53411138127));
#80984=CARTESIAN_POINT('Ctrl Pts',(16.7329911455468,-18.2608354603816,-16.5334021211097));
#80985=CARTESIAN_POINT('Ctrl Pts',(16.7305636178113,-18.2679038699715,-16.5329443592239));
#80986=CARTESIAN_POINT('Ctrl Pts',(16.7166116786433,-18.3092399734625,-16.5302602773391));
#80987=CARTESIAN_POINT('Ctrl Pts',(16.7059299249571,-18.3437833444819,-16.527988972574));
#80988=CARTESIAN_POINT('Ctrl Pts',(16.6743068167818,-18.4561679762689,-16.5205458836166));
#80989=CARTESIAN_POINT('Ctrl Pts',(16.6569252794185,-18.5349337236618,-16.5152498176493));
#80990=CARTESIAN_POINT('Ctrl Pts',(16.6261433829434,-18.725542196976,-16.5025015877908));
#80991=CARTESIAN_POINT('Ctrl Pts',(16.6170884083753,-18.8378502798878,-16.4950530971665));
#80992=CARTESIAN_POINT('Ctrl Pts',(16.6170006442199,-18.9503484472246,-16.4878149124144));
#80993=CARTESIAN_POINT('Ctrl Pts',(16.6170006421844,-18.950351058477,-16.4878147444052));
#80994=CARTESIAN_POINT('Ctrl Pts',(16.6169350225851,-19.0345970111522,-16.4823943227854));
#80995=CARTESIAN_POINT('Ctrl Pts',(16.6218981987577,-19.1187818305546,-16.4770994274566));
#80996=CARTESIAN_POINT('Ctrl Pts',(16.6330988071922,-19.2127900135317,-16.4713270383168));
#80997=CARTESIAN_POINT('Ctrl Pts',(16.6344059067415,-19.2231123433587,-16.470695060677));
#80998=CARTESIAN_POINT('Ctrl Pts',(16.6367383502125,-19.2405022784468,-16.4696333962698));
#80999=CARTESIAN_POINT('Ctrl Pts',(16.6377234421186,-19.2475750110736,-16.4692024471379));
#81000=CARTESIAN_POINT('Ctrl Pts',(16.6396009381099,-19.2605732900813,-16.4684119641199));
#81001=CARTESIAN_POINT('Ctrl Pts',(16.640482747474,-19.2665002707839,-16.4680520988851));
#81002=CARTESIAN_POINT('Ctrl Pts',(16.6423536700532,-19.27871882569,-16.4673114013629));
#81003=CARTESIAN_POINT('Ctrl Pts',(16.6433460343191,-19.2850098463914,-16.4669306761883));
#81004=CARTESIAN_POINT('Ctrl Pts',(16.6456303028236,-19.2990780301301,-16.4660806799525));
#81005=CARTESIAN_POINT('Ctrl Pts',(16.6469372952717,-19.306852673919,-16.4656118929438));
#81006=CARTESIAN_POINT('Ctrl Pts',(16.6503588008292,-19.3265324429957,-16.4644275862324));
#81007=CARTESIAN_POINT('Ctrl Pts',(16.6525319517493,-19.3384271871218,-16.4637139331016));
#81008=CARTESIAN_POINT('Ctrl Pts',(16.6655166180058,-19.4062088468947,-16.4596586362792));
#81009=CARTESIAN_POINT('Ctrl Pts',(16.6784773407092,-19.461663229567,-16.4563861926103));
#81010=CARTESIAN_POINT('Ctrl Pts',(16.7044778887797,-19.5556349278304,-16.4508783781244));
#81011=CARTESIAN_POINT('Ctrl Pts',(16.71641941116,-19.5944203584224,-16.4486161291037));
#81012=CARTESIAN_POINT('Ctrl Pts',(16.7346157472973,-19.6479940728282,-16.4454900620391));
#81013=CARTESIAN_POINT('Ctrl Pts',(16.7399331058666,-19.663085142709,-16.4446093145535));
#81014=CARTESIAN_POINT('Ctrl Pts',(16.7454194329591,-19.6781104106039,-16.4437313840672));
#81015=CARTESIAN_POINT('Origin',(18.734,-18.952,0.));
#81016=CARTESIAN_POINT('',(16.7454194499637,-19.6781104571738,-15.6464962048466));
#81017=CARTESIAN_POINT('',(16.7454194501832,-19.6781104577752,-15.8662164286365));
#81018=CARTESIAN_POINT('',(16.7454194499637,-19.6781104571739,0.));
#81019=CARTESIAN_POINT('Ctrl Pts',(16.7454194501833,-19.6781104577752,-15.8662164286365));
#81020=CARTESIAN_POINT('Ctrl Pts',(16.7372703347662,-19.6557926792016,-15.8675066642955));
#81021=CARTESIAN_POINT('Ctrl Pts',(16.7294937152069,-19.6333289218962,-15.8687972040221));
#81022=CARTESIAN_POINT('Ctrl Pts',(16.6950140071841,-19.5280200481297,-15.8748264318793));
#81023=CARTESIAN_POINT('Ctrl Pts',(16.6730620557294,-19.4437269241824,-15.8795907813764));
#81024=CARTESIAN_POINT('Ctrl Pts',(16.6490998720476,-19.3212039000817,-15.8867186533905));
#81025=CARTESIAN_POINT('Ctrl Pts',(16.6428359557392,-19.283892458455,-15.8889160472875));
#81026=CARTESIAN_POINT('Ctrl Pts',(16.6365221775586,-19.2389374853729,-15.8916169963615));
#81027=CARTESIAN_POINT('Ctrl Pts',(16.6355092983807,-19.2314335474448,-15.8920696192867));
#81028=CARTESIAN_POINT('Ctrl Pts',(16.633999500955,-19.2197767652956,-15.8927757145532));
#81029=CARTESIAN_POINT('Ctrl Pts',(16.6334745846423,-19.2156275227724,-15.893027635281));
#81030=CARTESIAN_POINT('Ctrl Pts',(16.632525166272,-19.2079398830612,-15.8934955182764));
#81031=CARTESIAN_POINT('Ctrl Pts',(16.6320973022205,-19.2044019592219,-15.893711288639));
#81032=CARTESIAN_POINT('Ctrl Pts',(16.6311517265553,-19.1964140123727,-15.8941994589649));
#81033=CARTESIAN_POINT('Ctrl Pts',(16.630639209231,-19.1919634421649,-15.8944721459476));
#81034=CARTESIAN_POINT('Ctrl Pts',(16.6291723812961,-19.1788600409237,-15.8952769781407));
#81035=CARTESIAN_POINT('Ctrl Pts',(16.6282573251611,-19.170203033916,-15.8958112514642));
#81036=CARTESIAN_POINT('Ctrl Pts',(16.6221408153505,-19.1087111158599,-15.8996231482018));
#81037=CARTESIAN_POINT('Ctrl Pts',(16.6188755553666,-19.0557070404166,-15.9029969230022));
#81038=CARTESIAN_POINT('Ctrl Pts',(16.6172125016367,-18.9862051693057,-15.9074892857674));
#81039=CARTESIAN_POINT('Ctrl Pts',(16.6170107020019,-18.9697651382934,-15.9085569565694));
#81040=CARTESIAN_POINT('Ctrl Pts',(16.6169886661743,-18.9345501864226,-15.910852690008));
#81041=CARTESIAN_POINT('Ctrl Pts',(16.6172266707935,-18.9157766073064,-15.9120819059916));
#81042=CARTESIAN_POINT('Ctrl Pts',(16.6217705414464,-18.7409093396794,-15.9235687458873));
#81043=CARTESIAN_POINT('Ctrl Pts',(16.6430867211467,-18.5857152159715,-15.9339904918105));
#81044=CARTESIAN_POINT('Ctrl Pts',(16.6824568347016,-18.4296182623915,-15.9442508982956));
#81045=CARTESIAN_POINT('Ctrl Pts',(16.6836465121877,-18.4249681087383,-15.9445563983091));
#81046=CARTESIAN_POINT('Ctrl Pts',(16.7007571342291,-18.359021806834,-15.9488865474276));
#81047=CARTESIAN_POINT('Ctrl Pts',(16.7194060610022,-18.2984617249976,-15.9528331782942));
#81048=CARTESIAN_POINT('Ctrl Pts',(16.7449593097039,-18.2270429779827,-15.9574536825387));
#81049=CARTESIAN_POINT('Ctrl Pts',(16.7492788043921,-18.2152996961582,-15.9582123647703));
#81050=CARTESIAN_POINT('Ctrl Pts',(16.7565350599576,-18.1960994629787,-15.9594512257848));
#81051=CARTESIAN_POINT('Ctrl Pts',(16.7594104544035,-18.1886197931944,-15.9599334418581));
#81052=CARTESIAN_POINT('Ctrl Pts',(16.7646512969167,-18.1752147095066,-15.9607970148743));
#81053=CARTESIAN_POINT('Ctrl Pts',(16.7670011814372,-18.1692833520257,-15.9611788887989));
#81054=CARTESIAN_POINT('Ctrl Pts',(16.772057444012,-18.1566873908091,-15.9619893893467));
#81055=CARTESIAN_POINT('Ctrl Pts',(16.7747710537981,-18.1500257624715,-15.9624177663289));
#81056=CARTESIAN_POINT('Ctrl Pts',(16.7821563599653,-18.1321568264676,-15.9635661745951));
#81057=CARTESIAN_POINT('Ctrl Pts',(16.7868906525702,-18.1209755582761,-15.9642840786211));
#81058=CARTESIAN_POINT('Ctrl Pts',(16.8108464004613,-18.0657265600386,-15.9678287044714));
#81059=CARTESIAN_POINT('Ctrl Pts',(16.8314697893408,-18.0222797762008,-15.9706071483523));
#81060=CARTESIAN_POINT('Ctrl Pts',(16.9305680820079,-17.8306476235727,-15.9828818136258));
#81061=CARTESIAN_POINT('Ctrl Pts',(17.0249942527189,-17.6914054106297,-15.9918000628666));
#81062=CARTESIAN_POINT('Ctrl Pts',(17.1995488648122,-17.4901881659197,-16.0063839563767));
#81063=CARTESIAN_POINT('Ctrl Pts',(17.2693656376801,-17.4202444105187,-16.0118767114489));
#81064=CARTESIAN_POINT('Ctrl Pts',(17.3511068420273,-17.3490684642471,-16.0182979722239));
#81065=CARTESIAN_POINT('Ctrl Pts',(17.3584620171353,-17.3427522737928,-16.0188757105727));
#81066=CARTESIAN_POINT('Ctrl Pts',(17.3693853966609,-17.3335015216189,-16.0197340934665));
#81067=CARTESIAN_POINT('Ctrl Pts',(17.3729203594835,-17.3305276593748,-16.0200119346769));
#81068=CARTESIAN_POINT('Ctrl Pts',(17.3792087461223,-17.3252724738799,-16.0205063471644));
#81069=CARTESIAN_POINT('Ctrl Pts',(17.3819582459784,-17.3229865313653,-16.0207225764601));
#81070=CARTESIAN_POINT('Ctrl Pts',(17.3878614410547,-17.3181038379143,-16.0211869573383));
#81071=CARTESIAN_POINT('Ctrl Pts',(17.3910168173919,-17.3155092854105,-16.021435255173));
#81072=CARTESIAN_POINT('Ctrl Pts',(17.399698555727,-17.3084126230133,-16.0221185876823));
#81073=CARTESIAN_POINT('Ctrl Pts',(17.4052401183606,-17.3039293147464,-16.022554939886));
#81074=CARTESIAN_POINT('Ctrl Pts',(17.4349422076825,-17.2801465205998,-16.0248942040046));
#81075=CARTESIAN_POINT('Ctrl Pts',(17.4594994307903,-17.2613512280133,-16.0268298884726));
#81076=CARTESIAN_POINT('Ctrl Pts',(17.5350662537209,-17.2060969594658,-16.0327692589338));
#81077=CARTESIAN_POINT('Ctrl Pts',(17.5872900996043,-17.1713611088715,-16.0368503751244));
#81078=CARTESIAN_POINT('Ctrl Pts',(17.7561738710654,-17.0695442561145,-16.0498093953593));
#81079=CARTESIAN_POINT('Ctrl Pts',(17.8777424301249,-17.011223934353,-16.0587750487683));
#81080=CARTESIAN_POINT('Ctrl Pts',(18.0423576790512,-16.95075353411,-16.0700684998409));
#81081=CARTESIAN_POINT('Ctrl Pts',(18.081089600638,-16.9377843096704,-16.0726704465894));
#81082=CARTESIAN_POINT('Ctrl Pts',(18.1665838574833,-16.911882489028,-16.0782894208243));
#81083=CARTESIAN_POINT('Ctrl Pts',(18.2134654252641,-16.8994199410769,-16.0812910304164));
#81084=CARTESIAN_POINT('Ctrl Pts',(18.2730119884972,-16.8857624391251,-16.0850068970682));
#81085=CARTESIAN_POINT('Ctrl Pts',(18.2853121758558,-16.8830565856138,-16.0857693651917));
#81086=CARTESIAN_POINT('Ctrl Pts',(18.3048443099977,-16.8789421958838,-16.0869722355475));
#81087=CARTESIAN_POINT('Ctrl Pts',(18.3120605770515,-16.8774614028735,-16.0874149431685));
#81088=CARTESIAN_POINT('Ctrl Pts',(18.3255227051634,-16.8747720953552,-16.0882377081858));
#81089=CARTESIAN_POINT('Ctrl Pts',(18.3317665494526,-16.8735540130042,-16.0886180672727));
#81090=CARTESIAN_POINT('Ctrl Pts',(18.3456487778405,-16.8709106933413,-16.0894610129257));
#81091=CARTESIAN_POINT('Ctrl Pts',(18.353289733302,-16.8694993230886,-16.0899231528547));
#81092=CARTESIAN_POINT('Ctrl Pts',(18.3755207956689,-16.8655194411239,-16.0912625317377));
#81093=CARTESIAN_POINT('Ctrl Pts',(18.3901304948097,-16.8630619342365,-16.092136239277));
#81094=CARTESIAN_POINT('Ctrl Pts',(18.5067618096874,-16.8447000700295,-16.0990618643436));
#81095=CARTESIAN_POINT('Ctrl Pts',(18.609803334359,-16.8361244369894,-16.1048707542409));
#81096=CARTESIAN_POINT('Ctrl Pts',(18.8727086928598,-16.8335251595991,-16.119346090252));
#81097=CARTESIAN_POINT('Ctrl Pts',(19.031997284835,-16.8500091641537,-16.1277744505008));
#81098=CARTESIAN_POINT('Ctrl Pts',(19.2353144808817,-16.8946403690136,-16.139529537776));
#81099=CARTESIAN_POINT('Ctrl Pts',(19.2823470765735,-16.9066737288974,-16.1423243045287));
#81100=CARTESIAN_POINT('Ctrl Pts',(19.3363662797182,-16.9224916708742,-16.1456660154322));
#81101=CARTESIAN_POINT('Ctrl Pts',(19.3437998689047,-16.9247128203816,-16.1461288035218));
#81102=CARTESIAN_POINT('Ctrl Pts',(19.3556666774905,-16.9283297841018,-16.1468725362401));
#81103=CARTESIAN_POINT('Ctrl Pts',(19.3601078802106,-16.9296994481504,-16.1471519938138));
#81104=CARTESIAN_POINT('Ctrl Pts',(19.3679699583758,-16.9321524889215,-16.1476487385434));
#81105=CARTESIAN_POINT('Ctrl Pts',(19.3713926319858,-16.9332299515151,-16.1478656771871));
#81106=CARTESIAN_POINT('Ctrl Pts',(19.3786461699568,-16.9355336615265,-16.1483269039742));
#81107=CARTESIAN_POINT('Ctrl Pts',(19.382476223875,-16.9367621070747,-16.1485713144113));
#81108=CARTESIAN_POINT('Ctrl Pts',(19.3928139944947,-16.9401103497302,-16.1492333172739));
#81109=CARTESIAN_POINT('Ctrl Pts',(19.3993149046837,-16.9422507820992,-16.1496520960965));
#81110=CARTESIAN_POINT('Ctrl Pts',(19.4316547552038,-16.9530728211618,-16.1517473431767));
#81111=CARTESIAN_POINT('Ctrl Pts',(19.4573334247137,-16.9622209627075,-16.1534491484479));
#81112=CARTESIAN_POINT('Ctrl Pts',(19.53124858766,-16.9901733847922,-16.1584445562623));
#81113=CARTESIAN_POINT('Ctrl Pts',(19.5789792332993,-17.0102537877554,-16.1617913664516));
#81114=CARTESIAN_POINT('Ctrl Pts',(19.7513269543476,-17.0903192847404,-16.174213526663));
#81115=CARTESIAN_POINT('Ctrl Pts',(19.8707327340156,-17.1607289522861,-16.1834600987806));
#81116=CARTESIAN_POINT('Ctrl Pts',(20.0600479526787,-17.2989648119022,-16.1986383744613));
#81117=CARTESIAN_POINT('Ctrl Pts',(20.133735067057,-17.3608762734982,-16.2047110354426));
#81118=CARTESIAN_POINT('Ctrl Pts',(20.2129592962322,-17.4372191776249,-16.2114253125287));
#81119=CARTESIAN_POINT('Ctrl Pts',(20.2228563068343,-17.4469456980767,-16.2122678406753));
#81120=CARTESIAN_POINT('Ctrl Pts',(20.238543465594,-17.4626688023455,-16.21360955599));
#81121=CARTESIAN_POINT('Ctrl Pts',(20.2443949460963,-17.4686033685904,-16.2141114590476));
#81122=CARTESIAN_POINT('Ctrl Pts',(20.2547039919481,-17.4791830354241,-16.2149983141814));
#81123=CARTESIAN_POINT('Ctrl Pts',(20.2591756726663,-17.483814176885,-16.2153838830514));
#81124=CARTESIAN_POINT('Ctrl Pts',(20.2684305113066,-17.4934869556387,-16.2161837635302));
#81125=CARTESIAN_POINT('Ctrl Pts',(20.2732101141948,-17.4985318989633,-16.21659791847));
#81126=CARTESIAN_POINT('Ctrl Pts',(20.2855195228238,-17.5116534802965,-16.2176673646747));
#81127=CARTESIAN_POINT('Ctrl Pts',(20.2930111963687,-17.5197657233853,-16.2183210173688));
#81128=CARTESIAN_POINT('Ctrl Pts',(20.3249207388038,-17.554865528277,-16.2211176600265));
#81129=CARTESIAN_POINT('Ctrl Pts',(20.3487048042152,-17.5824226353241,-16.2232339409861));
#81130=CARTESIAN_POINT('Ctrl Pts',(20.4096658827529,-17.6568513174003,-16.2287590731736));
#81131=CARTESIAN_POINT('Ctrl Pts',(20.4455879951238,-17.7047095012102,-16.2321204281713));
#81132=CARTESIAN_POINT('Ctrl Pts',(20.5743802826088,-17.892358956618,-16.2447295055551));
#81133=CARTESIAN_POINT('Ctrl Pts',(20.6525336174655,-18.0414727667594,-16.2535601340439));
#81134=CARTESIAN_POINT('Ctrl Pts',(20.7314610822797,-18.2486186819283,-16.2660208019192));
#81135=CARTESIAN_POINT('Ctrl Pts',(20.7487249397084,-18.29971292963,-16.2691133738655));
#81136=CARTESIAN_POINT('Ctrl Pts',(20.7664984314635,-18.3597875911247,-16.2728309766068));
#81137=CARTESIAN_POINT('Ctrl Pts',(20.7689263695775,-18.3681848960799,-16.273352453169));
#81138=CARTESIAN_POINT('Ctrl Pts',(20.7725219681294,-18.3809156580833,-16.2741461335582));
#81139=CARTESIAN_POINT('Ctrl Pts',(20.7737280018862,-18.3852383061664,-16.2744161605898));
#81140=CARTESIAN_POINT('Ctrl Pts',(20.7758672110919,-18.3930008977206,-16.2749020921806));
#81141=CARTESIAN_POINT('Ctrl Pts',(20.7768054513431,-18.3964393896689,-16.275117699115));
#81142=CARTESIAN_POINT('Ctrl Pts',(20.7788242308213,-18.403912135396,-16.2755870634525));
#81143=CARTESIAN_POINT('Ctrl Pts',(20.7799015026422,-18.4079471688606,-16.2758410008417));
#81144=CARTESIAN_POINT('Ctrl Pts',(20.7828913476432,-18.4192804043579,-16.2765555768137));
#81145=CARTESIAN_POINT('Ctrl Pts',(20.7847768338458,-18.4265855960734,-16.2770177357182));
#81146=CARTESIAN_POINT('Ctrl Pts',(20.795764778106,-18.4701179926372,-16.2797803932719));
#81147=CARTESIAN_POINT('Ctrl Pts',(20.8039455709976,-18.5065685165476,-16.2821289400003));
#81148=CARTESIAN_POINT('Ctrl Pts',(20.8276019738143,-18.6267732820587,-16.2899475036255));
#81149=CARTESIAN_POINT('Ctrl Pts',(20.8389884247766,-18.7112438844614,-16.2955549415315));
#81150=CARTESIAN_POINT('Ctrl Pts',(20.8583667167199,-18.9737803897779,-16.3129456621551));
#81151=CARTESIAN_POINT('Ctrl Pts',(20.849013248908,-19.1523790932572,-16.324649687209));
#81152=CARTESIAN_POINT('Ctrl Pts',(20.8133486346228,-19.3501424844108,-16.337016254709));
#81153=CARTESIAN_POINT('Ctrl Pts',(20.8089428419907,-19.3725002358559,-16.3384070518362));
#81154=CARTESIAN_POINT('Ctrl Pts',(20.8021872471084,-19.4040851641647,-16.3403621676895));
#81155=CARTESIAN_POINT('Ctrl Pts',(20.8001349855574,-19.4133737214395,-16.3409359426052));
#81156=CARTESIAN_POINT('Ctrl Pts',(20.7966949890208,-19.428459769655,-16.3418659862223));
#81157=CARTESIAN_POINT('Ctrl Pts',(20.7953452681792,-19.4342657113208,-16.3422234698676));
#81158=CARTESIAN_POINT('Ctrl Pts',(20.7924655870635,-19.4464199294729,-16.3429709193507));
#81159=CARTESIAN_POINT('Ctrl Pts',(20.7909307379732,-19.452766992162,-16.3433607234993));
#81160=CARTESIAN_POINT('Ctrl Pts',(20.7872036394685,-19.4678733798395,-16.3442872848735));
#81161=CARTESIAN_POINT('Ctrl Pts',(20.7849846575012,-19.4766260265132,-16.3448231740085));
#81162=CARTESIAN_POINT('Ctrl Pts',(20.7772910205284,-19.5061781139872,-16.3466294806816));
#81163=CARTESIAN_POINT('Ctrl Pts',(20.7715553129258,-19.5269086653753,-16.3478914522964));
#81164=CARTESIAN_POINT('Ctrl Pts',(20.7148921410049,-19.72019507986,-16.3596187548537));
#81165=CARTESIAN_POINT('Ctrl Pts',(20.6424810743416,-19.885683184866,-16.3692827107052));
#81166=CARTESIAN_POINT('Ctrl Pts',(20.4883353213915,-20.1429637841121,-16.3856069446835));
#81167=CARTESIAN_POINT('Ctrl Pts',(20.4180341199188,-20.2404517273013,-16.3921921004463));
#81168=CARTESIAN_POINT('Ctrl Pts',(20.3336708919768,-20.3386623697774,-16.399865070986));
#81169=CARTESIAN_POINT('Ctrl Pts',(20.3274239761863,-20.3458362582712,-16.4004320763371));
#81170=CARTESIAN_POINT('Ctrl Pts',(20.3180955402748,-20.3564042622438,-16.4012774942516));
#81171=CARTESIAN_POINT('Ctrl Pts',(20.3150509023666,-20.3598309755598,-16.4015532242197));
#81172=CARTESIAN_POINT('Ctrl Pts',(20.3096138989233,-20.3659103938445,-16.4020453159078));
#81173=CARTESIAN_POINT('Ctrl Pts',(20.307225925006,-20.36856695887,-16.4022613476075));
#81174=CARTESIAN_POINT('Ctrl Pts',(20.3020771778445,-20.3742657419567,-16.4027269410849));
#81175=CARTESIAN_POINT('Ctrl Pts',(20.2993143103751,-20.377305926983,-16.4029766577034));
#81176=CARTESIAN_POINT('Ctrl Pts',(20.2916630066476,-20.3856761363734,-16.4036678129278));
#81177=CARTESIAN_POINT('Ctrl Pts',(20.2867561323809,-20.3909891230169,-16.4041106186315));
#81178=CARTESIAN_POINT('Ctrl Pts',(20.2597168805611,-20.419966916857,-16.4065477680321));
#81179=CARTESIAN_POINT('Ctrl Pts',(20.2370719402452,-20.4431449778755,-16.4085781475792));
#81180=CARTESIAN_POINT('Ctrl Pts',(20.0974804802588,-20.579611596734,-16.4209812558022));
#81181=CARTESIAN_POINT('Ctrl Pts',(19.9683173785099,-20.679616581074,-16.4319460768));
#81182=CARTESIAN_POINT('Ctrl Pts',(19.7289709719092,-20.8242644031252,-16.4502135242569));
#81183=CARTESIAN_POINT('Ctrl Pts',(19.6241275051833,-20.8763237946651,-16.4576564611517));
#81184=CARTESIAN_POINT('Ctrl Pts',(19.5022239938354,-20.9247455896178,-16.4656656227366));
#81185=CARTESIAN_POINT('Ctrl Pts',(19.488887991633,-20.9298871054424,-16.4665337725271));
#81186=CARTESIAN_POINT('Ctrl Pts',(19.4675809751566,-20.9378548399909,-16.4679083033623));
#81187=CARTESIAN_POINT('Ctrl Pts',(19.459643508529,-20.94076896456,-16.4684176139481));
#81188=CARTESIAN_POINT('Ctrl Pts',(19.4456142137588,-20.9458244410496,-16.4693130502426));
#81189=CARTESIAN_POINT('Ctrl Pts',(19.4395296886263,-20.9479856088786,-16.4696998323463));
#81190=CARTESIAN_POINT('Ctrl Pts',(19.4269249371902,-20.9523978629374,-16.4704978900684));
#81191=CARTESIAN_POINT('Ctrl Pts',(19.4204033985751,-20.9546449897025,-16.4709090304463));
#81192=CARTESIAN_POINT('Ctrl Pts',(19.4036362611302,-20.9603309169603,-16.4719616317673));
#81193=CARTESIAN_POINT('Ctrl Pts',(19.3933750221711,-20.9637232366635,-16.4726015520328));
#81194=CARTESIAN_POINT('Ctrl Pts',(19.3504477926322,-20.9775510502206,-16.4752613566935));
#81195=CARTESIAN_POINT('Ctrl Pts',(19.3175555766062,-20.9872709950973,-16.4772577317778));
#81196=CARTESIAN_POINT('Ctrl Pts',(19.2312587072101,-21.0105082290224,-16.4823994315742));
#81197=CARTESIAN_POINT('Ctrl Pts',(19.1775361357973,-21.0227483409673,-16.4855054150318));
#81198=CARTESIAN_POINT('Ctrl Pts',(19.0159372518612,-21.0529882753304,-16.4946470768221));
#81199=CARTESIAN_POINT('Ctrl Pts',(18.9070811406451,-21.0647432764596,-16.500534016658));
#81200=CARTESIAN_POINT('Ctrl Pts',(18.754557487999,-21.0693422957247,-16.5088416995531));
#81201=CARTESIAN_POINT('Ctrl Pts',(18.7112817142969,-21.0693201676826,-16.5112068805828));
#81202=CARTESIAN_POINT('Ctrl Pts',(18.5928022414449,-21.0656267771603,-16.5177700317084));
#81203=CARTESIAN_POINT('Ctrl Pts',(18.5177529915108,-21.0592706621016,-16.5220240790493));
#81204=CARTESIAN_POINT('Ctrl Pts',(18.433813817885,-21.047630514903,-16.527046539221));
#81205=CARTESIAN_POINT('Ctrl Pts',(18.4244260268215,-21.0462642971886,-16.5276120225052));
#81206=CARTESIAN_POINT('Ctrl Pts',(18.4105213361184,-21.0441451957291,-16.528455600293));
#81207=CARTESIAN_POINT('Ctrl Pts',(18.4059970370115,-21.0434406569076,-16.5287310291195));
#81208=CARTESIAN_POINT('Ctrl Pts',(18.3979477694756,-21.0421604376735,-16.529222791435));
#81209=CARTESIAN_POINT('Ctrl Pts',(18.3944219373657,-21.0415905091673,-16.5294387966109));
#81210=CARTESIAN_POINT('Ctrl Pts',(18.3868404097546,-21.0403453074201,-16.5299045706142));
#81211=CARTESIAN_POINT('Ctrl Pts',(18.382785293564,-21.0396671510185,-16.5301544955373));
#81212=CARTESIAN_POINT('Ctrl Pts',(18.3715873651308,-21.0377609187876,-16.5308468012469));
#81213=CARTESIAN_POINT('Ctrl Pts',(18.3644489230377,-21.03650798182,-16.5312905564889));
#81214=CARTESIAN_POINT('Ctrl Pts',(18.3252118006344,-21.0294132144889,-16.5337425227298));
#81215=CARTESIAN_POINT('Ctrl Pts',(18.2932469065661,-21.0228669428704,-16.5357872775799));
#81216=CARTESIAN_POINT('Ctrl Pts',(18.102923303442,-20.9792836830192,-16.5481952218939));
#81217=CARTESIAN_POINT('Ctrl Pts',(17.9491137172016,-20.9248381569016,-16.5591468745221));
#81218=CARTESIAN_POINT('Ctrl Pts',(17.698177629127,-20.8019721539079,-16.5773969993904));
#81219=CARTESIAN_POINT('Ctrl Pts',(17.5977167085537,-20.742025987069,-16.5848353319221));
#81220=CARTESIAN_POINT('Ctrl Pts',(17.4910707202066,-20.6657736644029,-16.5928404902917));
#81221=CARTESIAN_POINT('Ctrl Pts',(17.4795260775724,-20.6573411861138,-16.5937088582423));
#81222=CARTESIAN_POINT('Ctrl Pts',(17.4612896724176,-20.6437354793409,-16.595083668108));
#81223=CARTESIAN_POINT('Ctrl Pts',(17.4545421187629,-20.6386380890332,-16.595593041415));
#81224=CARTESIAN_POINT('Ctrl Pts',(17.4426964996947,-20.6295774090116,-16.5964885506709));
#81225=CARTESIAN_POINT('Ctrl Pts',(17.437585718763,-20.6256309945637,-16.5968753433513));
#81226=CARTESIAN_POINT('Ctrl Pts',(17.427224592324,-20.6175544589851,-16.5976603990638));
#81227=CARTESIAN_POINT('Ctrl Pts',(17.4219755768825,-20.6134227447185,-16.5980585927475));
#81228=CARTESIAN_POINT('Ctrl Pts',(17.408667114926,-20.6028447081675,-16.5990694635341));
#81229=CARTESIAN_POINT('Ctrl Pts',(17.4006350297258,-20.5963641228461,-16.5996807631242));
#81230=CARTESIAN_POINT('Ctrl Pts',(17.3833150813318,-20.5821793938909,-16.6010017738933));
#81231=CARTESIAN_POINT('Ctrl Pts',(17.3740450171815,-20.574454023816,-16.601710610031));
#81232=CARTESIAN_POINT('Ctrl Pts',(17.3475939408034,-20.5520245645737,-16.603738896327));
#81233=CARTESIAN_POINT('Ctrl Pts',(17.330581512773,-20.5371236460894,-16.6050504224965));
#81234=CARTESIAN_POINT('Ctrl Pts',(17.2733864095188,-20.4853845817584,-16.6094885618791));
#81235=CARTESIAN_POINT('Ctrl Pts',(17.2343878027962,-20.4472672744546,-16.6125639234843));
#81236=CARTESIAN_POINT('Ctrl Pts',(17.1220538027896,-20.3286506781454,-16.6216521111689));
#81237=CARTESIAN_POINT('Ctrl Pts',(17.0534107792096,-20.2439591491638,-16.6275160339473));
#81238=CARTESIAN_POINT('Ctrl Pts',(16.9234840216056,-20.0556749204459,-16.639967260909));
#81239=CARTESIAN_POINT('Ctrl Pts',(16.8638998360526,-19.9513915378515,-16.6465480302672));
#81240=CARTESIAN_POINT('Ctrl Pts',(16.8094654177348,-19.8340125791549,-16.6542160209437));
#81241=CARTESIAN_POINT('Ctrl Pts',(16.8055204012333,-19.8253532948458,-16.6547832048003));
#81242=CARTESIAN_POINT('Ctrl Pts',(16.799761470724,-19.8124831955633,-16.6556288384967));
#81243=CARTESIAN_POINT('Ctrl Pts',(16.7979025800113,-19.8082924718744,-16.6559046037539));
#81244=CARTESIAN_POINT('Ctrl Pts',(16.794619514984,-19.8008257153549,-16.656396734067));
#81245=CARTESIAN_POINT('Ctrl Pts',(16.7931900054604,-19.7975520833015,-16.6566127689027));
#81246=CARTESIAN_POINT('Ctrl Pts',(16.790134469513,-19.7905062149881,-16.657078341352));
#81247=CARTESIAN_POINT('Ctrl Pts',(16.7885111584007,-19.7867329152124,-16.6573280336598));
#81248=CARTESIAN_POINT('Ctrl Pts',(16.7840607654319,-19.776304714235,-16.6580190546477));
#81249=CARTESIAN_POINT('Ctrl Pts',(16.7812568114658,-19.7696400898785,-16.6584617495682));
#81250=CARTESIAN_POINT('Ctrl Pts',(16.7668566461675,-19.7349162288726,-16.6607733010531));
#81251=CARTESIAN_POINT('Ctrl Pts',(16.7558316161175,-19.7066259962242,-16.6626735717684));
#81252=CARTESIAN_POINT('Ctrl Pts',(16.7454194499739,-19.6781104572019,-16.6645989847956));
#81253=CARTESIAN_POINT('Ctrl Pts',(16.7454194329591,-19.6781104106039,-16.4437313840672));
#81254=CARTESIAN_POINT('Ctrl Pts',(16.790870432835,-19.8025859363448,-16.4364582452718));
#81255=CARTESIAN_POINT('Ctrl Pts',(16.8479181674973,-19.9225464740244,-16.4293983430912));
#81256=CARTESIAN_POINT('Ctrl Pts',(16.9473167103501,-20.0892030165193,-16.4185943673103));
#81257=CARTESIAN_POINT('Ctrl Pts',(16.9810870901895,-20.1405969870292,-16.4151048852973));
#81258=CARTESIAN_POINT('Ctrl Pts',(17.0245020075486,-20.200786707114,-16.4107315787639));
#81259=CARTESIAN_POINT('Ctrl Pts',(17.0320553064698,-20.2110615029907,-16.4099744760412));
#81260=CARTESIAN_POINT('Ctrl Pts',(17.042796460597,-20.2253994847967,-16.4089020906605));
#81261=CARTESIAN_POINT('Ctrl Pts',(17.0459072301081,-20.2295204337018,-16.4085920048467));
#81262=CARTESIAN_POINT('Ctrl Pts',(17.051248104375,-20.236542115058,-16.4080603741517));
#81263=CARTESIAN_POINT('Ctrl Pts',(17.0534707368775,-20.2394485555461,-16.4078393537839));
#81264=CARTESIAN_POINT('Ctrl Pts',(17.0577587450601,-20.2450257746831,-16.4074133441053));
#81265=CARTESIAN_POINT('Ctrl Pts',(17.0598229851405,-20.2476973880126,-16.4072084395794));
#81266=CARTESIAN_POINT('Ctrl Pts',(17.0653347550376,-20.2547957560812,-16.4066618124772));
#81267=CARTESIAN_POINT('Ctrl Pts',(17.068793479839,-20.2592137259725,-16.4063193047755));
#81268=CARTESIAN_POINT('Ctrl Pts',(17.0812698832623,-20.2750204779662,-16.4050857823426));
#81269=CARTESIAN_POINT('Ctrl Pts',(17.0903869325908,-20.2863298250179,-16.4041880754989));
#81270=CARTESIAN_POINT('Ctrl Pts',(17.2005041091458,-20.4200849236513,-16.3933978926925));
#81271=CARTESIAN_POINT('Ctrl Pts',(17.3148424589957,-20.5308821178171,-16.3827536433332));
#81272=CARTESIAN_POINT('Ctrl Pts',(17.5176071082078,-20.6873877011818,-16.3658986061808));
#81273=CARTESIAN_POINT('Ctrl Pts',(17.5987614499756,-20.7415304798629,-16.3595729150787));
#81274=CARTESIAN_POINT('Ctrl Pts',(17.7122871256008,-20.8064275698765,-16.3513404788038));
#81275=CARTESIAN_POINT('Ctrl Pts',(17.741596230581,-20.8222763863991,-16.3492657415093));
#81276=CARTESIAN_POINT('Ctrl Pts',(17.7854580167468,-20.8446729626536,-16.3462342720938));
#81277=CARTESIAN_POINT('Ctrl Pts',(17.799729144325,-20.851758097113,-16.3452591350037));
#81278=CARTESIAN_POINT('Ctrl Pts',(17.8257480175641,-20.86431147907,-16.3435012080746));
#81279=CARTESIAN_POINT('Ctrl Pts',(17.8374684592054,-20.8698342119811,-16.3427165589774));
#81280=CARTESIAN_POINT('Ctrl Pts',(17.8559006557477,-20.8783136582262,-16.3414936641234));
#81281=CARTESIAN_POINT('Ctrl Pts',(17.8625781826974,-20.8813436155032,-16.3410528970905));
#81282=CARTESIAN_POINT('Ctrl Pts',(17.8693098683501,-20.8843560691563,-16.3406107948684));
#81283=CARTESIAN_POINT('Ctrl Pts',(17.8693483533328,-20.8843732899451,-16.3406082674477));
#81284=CARTESIAN_POINT('Ctrl Pts',(17.8694266528058,-20.8844083236273,-16.340603125443));
#81285=CARTESIAN_POINT('Ctrl Pts',(17.8694664677064,-20.8844261366072,-16.3406005108372));
#81286=CARTESIAN_POINT('Ctrl Pts',(17.8695474765426,-20.8844623765354,-16.3405951912257));
#81287=CARTESIAN_POINT('Ctrl Pts',(17.8695886703042,-20.8844808033018,-16.3405924862369));
#81288=CARTESIAN_POINT('Ctrl Pts',(17.8696724882164,-20.8845182934591,-16.3405869825039));
#81289=CARTESIAN_POINT('Ctrl Pts',(17.8697151123922,-20.8845373567497,-16.340584183764));
#81290=CARTESIAN_POINT('Ctrl Pts',(17.8698018534751,-20.8845761474981,-16.3405784884534));
#81291=CARTESIAN_POINT('Ctrl Pts',(17.8698459568872,-20.8845958688004,-16.3405755927754));
#81292=CARTESIAN_POINT('Ctrl Pts',(17.8699357066387,-20.8846359976562,-16.3405697003117));
#81293=CARTESIAN_POINT('Ctrl Pts',(17.869981354246,-20.884656405647,-16.3405667034499));
#81294=CARTESIAN_POINT('Ctrl Pts',(17.8700742454782,-20.8846979312222,-16.3405606051544));
#81295=CARTESIAN_POINT('Ctrl Pts',(17.8701214901366,-20.8847190491308,-16.3405575036602));
#81296=CARTESIAN_POINT('Ctrl Pts',(17.8702176357682,-20.884762021075,-16.3405511921638));
#81297=CARTESIAN_POINT('Ctrl Pts',(17.8702665377603,-20.8847838754179,-16.3405479821027));
#81298=CARTESIAN_POINT('Ctrl Pts',(17.8703660607466,-20.8848283477957,-16.3405414493814));
#81299=CARTESIAN_POINT('Ctrl Pts',(17.8704166827655,-20.8848509661294,-16.3405381266624));
#81300=CARTESIAN_POINT('Ctrl Pts',(17.8705197111997,-20.8848969952243,-16.3405313643588));
#81301=CARTESIAN_POINT('Ctrl Pts',(17.8705721184478,-20.8849204061864,-16.3405279247286));
#81302=CARTESIAN_POINT('Ctrl Pts',(17.8706787853405,-20.8849680503954,-16.3405209241672));
#81303=CARTESIAN_POINT('Ctrl Pts',(17.870733045853,-20.8849922838461,-16.3405173631887));
#81304=CARTESIAN_POINT('Ctrl Pts',(17.8708434900583,-20.8850416040868,-16.3405101153149));
#81305=CARTESIAN_POINT('Ctrl Pts',(17.8708996745735,-20.8850666910467,-16.3405064283761));
#81306=CARTESIAN_POINT('Ctrl Pts',(17.8710140406351,-20.885117750681,-16.3404989237674));
#81307=CARTESIAN_POINT('Ctrl Pts',(17.8710722227819,-20.8851437234113,-16.3404951060694));
#81308=CARTESIAN_POINT('Ctrl Pts',(17.871190660852,-20.8851965882011,-16.3404873349406));
#81309=CARTESIAN_POINT('Ctrl Pts',(17.8712509174634,-20.8852234803395,-16.3404833814768));
#81310=CARTESIAN_POINT('Ctrl Pts',(17.871373584344,-20.8852782189024,-16.3404753336124));
#81311=CARTESIAN_POINT('Ctrl Pts',(17.8714359952802,-20.8853060653792,-16.340471239181));
#81312=CARTESIAN_POINT('Ctrl Pts',(17.8715630540712,-20.8853627490224,-16.3404629039587));
#81313=CARTESIAN_POINT('Ctrl Pts',(17.8716277024957,-20.885391586179,-16.3404586631444));
#81314=CARTESIAN_POINT('Ctrl Pts',(17.871759322882,-20.885450289017,-16.3404500295168));
#81315=CARTESIAN_POINT('Ctrl Pts',(17.8718262954497,-20.8854801546846,-16.3404456366788));
#81316=CARTESIAN_POINT('Ctrl Pts',(17.8719626562509,-20.885540954765,-16.3404366930068));
#81317=CARTESIAN_POINT('Ctrl Pts',(17.8720320421291,-20.8855718878217,-16.3404321423436));
#81318=CARTESIAN_POINT('Ctrl Pts',(17.8721601038573,-20.8856289710135,-16.3404237438717));
#81319=CARTESIAN_POINT('Ctrl Pts',(17.8722187806341,-20.8856551228372,-16.3404198959346));
#81320=CARTESIAN_POINT('Ctrl Pts',(17.8723460084028,-20.8857118204108,-16.3404115528925));
#81321=CARTESIAN_POINT('Ctrl Pts',(17.8724145607914,-20.8857423656154,-16.340407057758));
#81322=CARTESIAN_POINT('Ctrl Pts',(17.8725632119349,-20.8858085913183,-16.3403973108709));
#81323=CARTESIAN_POINT('Ctrl Pts',(17.872643312163,-20.8858442708779,-16.3403920591065));
#81324=CARTESIAN_POINT('Ctrl Pts',(17.8728170160953,-20.8859216320037,-16.3403806709104));
#81325=CARTESIAN_POINT('Ctrl Pts',(17.8729106212553,-20.8859633120389,-16.340374534499));
#81326=CARTESIAN_POINT('Ctrl Pts',(17.8731136254053,-20.8860536870461,-16.3403612272282));
#81327=CARTESIAN_POINT('Ctrl Pts',(17.8732230259628,-20.8861023797377,-16.3403540564243));
#81328=CARTESIAN_POINT('Ctrl Pts',(17.8734603006058,-20.886207963316,-16.3403385052251));
#81329=CARTESIAN_POINT('Ctrl Pts',(17.8735881758082,-20.8862648506291,-16.3403301249728));
#81330=CARTESIAN_POINT('Ctrl Pts',(17.8738616666911,-20.8863864849013,-16.340312203577));
#81331=CARTESIAN_POINT('Ctrl Pts',(17.8740072841099,-20.8864512281296,-16.3403026625587));
#81332=CARTESIAN_POINT('Ctrl Pts',(17.8800535644706,-20.8891386583196,-16.3399065468012));
#81333=CARTESIAN_POINT('Ctrl Pts',(17.8859662385224,-20.8917343728278,-16.3395208998026));
#81334=CARTESIAN_POINT('Ctrl Pts',(17.8996506613505,-20.8976674218847,-16.338632259072));
#81335=CARTESIAN_POINT('Ctrl Pts',(17.9074307519843,-20.9009853300859,-16.338129932466));
#81336=CARTESIAN_POINT('Ctrl Pts',(17.9284186390258,-20.9097875745876,-16.3367824802344));
#81337=CARTESIAN_POINT('Ctrl Pts',(17.9416626125614,-20.9151849112528,-16.3359403018445));
#81338=CARTESIAN_POINT('Ctrl Pts',(18.0636053365809,-20.9634453736655,-16.3282574841005));
#81339=CARTESIAN_POINT('Ctrl Pts',(18.1756298754291,-20.9973776089088,-16.3217335538499));
#81340=CARTESIAN_POINT('Ctrl Pts',(18.4491388267183,-21.0560600675816,-16.3064198250329));
#81341=CARTESIAN_POINT('Ctrl Pts',(18.6117726556967,-21.0717318756183,-16.2978135107385));
#81342=CARTESIAN_POINT('Ctrl Pts',(18.8069306832055,-21.0679909046237,-16.2866039925212));
#81343=CARTESIAN_POINT('Ctrl Pts',(18.8392677397602,-21.066628770721,-16.2847161910742));
#81344=CARTESIAN_POINT('Ctrl Pts',(18.878773225667,-21.0640563395597,-16.2823589638163));
#81345=CARTESIAN_POINT('Ctrl Pts',(18.8859850599166,-21.0635496220732,-16.2819265636368));
#81346=CARTESIAN_POINT('Ctrl Pts',(18.8972899233484,-21.0626971058423,-16.2812452948227));
#81347=CARTESIAN_POINT('Ctrl Pts',(18.9013848606183,-21.0623763122852,-16.2809978071314));
#81348=CARTESIAN_POINT('Ctrl Pts',(18.9090393193728,-21.0617542505493,-16.2805338143156));
#81349=CARTESIAN_POINT('Ctrl Pts',(18.9125990207231,-21.0614558896018,-16.2803174737478));
#81350=CARTESIAN_POINT('Ctrl Pts',(18.9207257494407,-21.0607540195608,-16.2798223002071));
#81351=CARTESIAN_POINT('Ctrl Pts',(18.9252922161545,-21.060344684259,-16.2795431442299));
#81352=CARTESIAN_POINT('Ctrl Pts',(18.9393335414826,-21.059040035636,-16.2786820358269));
#81353=CARTESIAN_POINT('Ctrl Pts',(18.9488035686918,-21.0580956754469,-16.278097433364));
#81354=CARTESIAN_POINT('Ctrl Pts',(19.0774789355211,-21.0443871717375,-16.2701048129342));
#81355=CARTESIAN_POINT('Ctrl Pts',(19.1953834914841,-21.0215846132481,-16.2622176741382));
#81356=CARTESIAN_POINT('Ctrl Pts',(19.484144606796,-20.9398287306077,-16.2423911049925));
#81357=CARTESIAN_POINT('Ctrl Pts',(19.6506363054677,-20.8687638327228,-16.2305530386383));
#81358=CARTESIAN_POINT('Ctrl Pts',(19.824503642287,-20.7666473678887,-16.2181683321501));
#81359=CARTESIAN_POINT('Ctrl Pts',(19.8427182067667,-20.7555762400712,-16.2168692632026));
#81360=CARTESIAN_POINT('Ctrl Pts',(19.8683794335763,-20.7394432128729,-16.2150361647547));
#81361=CARTESIAN_POINT('Ctrl Pts',(19.875965344941,-20.7346062642732,-16.2144938950286));
#81362=CARTESIAN_POINT('Ctrl Pts',(19.8889986750243,-20.7261785768464,-16.2135615009464));
#81363=CARTESIAN_POINT('Ctrl Pts',(19.8944607080641,-20.7226107726902,-16.213170530257));
#81364=CARTESIAN_POINT('Ctrl Pts',(19.9048871161495,-20.7157312640052,-16.2124237498338));
#81365=CARTESIAN_POINT('Ctrl Pts',(19.9098541437289,-20.7124237115515,-16.212067789564));
#81366=CARTESIAN_POINT('Ctrl Pts',(19.922733333768,-20.7037686085051,-16.2111442379887));
#81367=CARTESIAN_POINT('Ctrl Pts',(19.9306234724815,-20.6983884064559,-16.2105778839342));
#81368=CARTESIAN_POINT('Ctrl Pts',(19.9574020030513,-20.6798617205987,-16.2086535479297));
#81369=CARTESIAN_POINT('Ctrl Pts',(19.9761127357752,-20.6664604397004,-16.2073052758252));
#81370=CARTESIAN_POINT('Ctrl Pts',(20.1353308296661,-20.5484478765306,-16.1957892854875));
#81371=CARTESIAN_POINT('Ctrl Pts',(20.2625690373503,-20.4270787534546,-16.1863693519422));
#81372=CARTESIAN_POINT('Ctrl Pts',(20.4285946627165,-20.2238668941518,-16.1720920257346));
#81373=CARTESIAN_POINT('Ctrl Pts',(20.4795474567863,-20.152982154557,-16.1673177413224));
#81374=CARTESIAN_POINT('Ctrl Pts',(20.5461470359653,-20.0471013030606,-16.1601764776963));
#81375=CARTESIAN_POINT('Ctrl Pts',(20.5654490634911,-20.0145053745493,-16.1579763405716));
#81376=CARTESIAN_POINT('Ctrl Pts',(20.5875483766073,-19.9747926445354,-16.1552723510711));
#81377=CARTESIAN_POINT('Ctrl Pts',(20.5911960988069,-19.9681540359541,-16.1548195644448));
#81378=CARTESIAN_POINT('Ctrl Pts',(20.5968027001453,-19.9578193661804,-16.1541132684264));
#81379=CARTESIAN_POINT('Ctrl Pts',(20.5987864265803,-19.9541367569344,-16.153861312065));
#81380=CARTESIAN_POINT('Ctrl Pts',(20.602439980852,-19.9473058515472,-16.153393396742));
#81381=CARTESIAN_POINT('Ctrl Pts',(20.6041127782342,-19.9441592091365,-16.153177629902));
#81382=CARTESIAN_POINT('Ctrl Pts',(20.6078702097987,-19.9370479685832,-16.1526895110134));
#81383=CARTESIAN_POINT('Ctrl Pts',(20.6099501990588,-19.9330809922625,-16.1524168722143));
#81384=CARTESIAN_POINT('Ctrl Pts',(20.6160338566233,-19.9213880967619,-16.1516123109474));
#81385=CARTESIAN_POINT('Ctrl Pts',(20.6200024410146,-19.9136441681554,-16.1510782624641));
#81386=CARTESIAN_POINT('Ctrl Pts',(20.647813158319,-19.8585425525057,-16.1472709083415));
#81387=CARTESIAN_POINT('Ctrl Pts',(20.669914486368,-19.8103322703828,-16.1439017005862));
#81388=CARTESIAN_POINT('Ctrl Pts',(20.6974113780925,-19.7438727332394,-16.1392543754242));
#81389=CARTESIAN_POINT('Ctrl Pts',(20.704406976404,-19.7263016096593,-16.138025381011));
#81390=CARTESIAN_POINT('Ctrl Pts',(20.7281751076773,-19.6641933764022,-16.1336853322327));
#81391=CARTESIAN_POINT('Ctrl Pts',(20.7436801987438,-19.6191874117372,-16.130547938903));
#81392=CARTESIAN_POINT('Ctrl Pts',(20.7897744966679,-19.4691484961866,-16.1201795930754));
#81393=CARTESIAN_POINT('Ctrl Pts',(20.8137458529611,-19.3622584568169,-16.1129475375456));
#81394=CARTESIAN_POINT('Ctrl Pts',(20.8372084631734,-19.1994630648936,-16.1023754510687));
#81395=CARTESIAN_POINT('Ctrl Pts',(20.8429360692748,-19.1446480841279,-16.0988870377518));
#81396=CARTESIAN_POINT('Ctrl Pts',(20.8487493920924,-19.0554426046535,-16.0933304857184));
#81397=CARTESIAN_POINT('Ctrl Pts',(20.8501478170604,-19.021166439767,-16.0912239257994));
#81398=CARTESIAN_POINT('Ctrl Pts',(20.8508908246223,-18.9760633851422,-16.0884877302167));
#81399=CARTESIAN_POINT('Ctrl Pts',(20.8509860899126,-18.9652556318372,-16.0878347603344));
#81400=CARTESIAN_POINT('Ctrl Pts',(20.8510065598869,-18.9475495836587,-16.0867693026503));
#81401=CARTESIAN_POINT('Ctrl Pts',(20.8509808212093,-18.9406516435527,-16.0863552856376));
#81402=CARTESIAN_POINT('Ctrl Pts',(20.8508657181623,-18.9272973407832,-16.0855557752481));
#81403=CARTESIAN_POINT('Ctrl Pts',(20.8507805294708,-18.920841027263,-16.0851701555803));
#81404=CARTESIAN_POINT('Ctrl Pts',(20.8505155760219,-18.9059315463767,-16.0842817146317));
#81405=CARTESIAN_POINT('Ctrl Pts',(20.8503147050802,-18.8974788280797,-16.0837795595154));
#81406=CARTESIAN_POINT('Ctrl Pts',(20.849638101385,-18.8747429523219,-16.082432870961));
#81407=CARTESIAN_POINT('Ctrl Pts',(20.8490683671309,-18.8604628778926,-16.0815912794742));
#81408=CARTESIAN_POINT('Ctrl Pts',(20.8425104977684,-18.7294206390747,-16.0739047929736));
#81409=CARTESIAN_POINT('Ctrl Pts',(20.8270039789032,-18.6133295019638,-16.0673770411299));
#81410=CARTESIAN_POINT('Ctrl Pts',(20.7671093396643,-18.339844901842,-16.0520508208194));
#81411=CARTESIAN_POINT('Ctrl Pts',(20.7139571800078,-18.1851720940548,-16.0434362593785));
#81412=CARTESIAN_POINT('Ctrl Pts',(20.6297096594212,-18.0091272720831,-16.0322260260118));
#81413=CARTESIAN_POINT('Ctrl Pts',(20.6151625807948,-17.9804284973649,-16.0303490608423));
#81414=CARTESIAN_POINT('Ctrl Pts',(20.5965595767998,-17.9457133105134,-16.0280038914757));
#81415=CARTESIAN_POINT('Ctrl Pts',(20.5931185269444,-17.9393700686196,-16.0275722674848));
#81416=CARTESIAN_POINT('Ctrl Pts',(20.5876695288222,-17.9294467613557,-16.0268919523945));
#81417=CARTESIAN_POINT('Ctrl Pts',(20.5856834486021,-17.9258546626033,-16.0266446358606));
#81418=CARTESIAN_POINT('Ctrl Pts',(20.5819491622501,-17.9191468362812,-16.0261807873233));
#81419=CARTESIAN_POINT('Ctrl Pts',(20.580203511372,-17.9160297504265,-16.0259644188014));
#81420=CARTESIAN_POINT('Ctrl Pts',(20.5761974743839,-17.9089187346331,-16.0254689478649));
#81421=CARTESIAN_POINT('Ctrl Pts',(20.5739319938753,-17.9049277399415,-16.0251895209438));
#81422=CARTESIAN_POINT('Ctrl Pts',(20.567981938688,-17.8945247336758,-16.0244576980905));
#81423=CARTESIAN_POINT('Ctrl Pts',(20.564276747183,-17.8881246711347,-16.024004021211));
#81424=CARTESIAN_POINT('Ctrl Pts',(20.5397061299632,-17.8461915439389,-16.0210094648727));
#81425=CARTESIAN_POINT('Ctrl Pts',(20.5178420378848,-17.811257243094,-16.0184102381458));
#81426=CARTESIAN_POINT('Ctrl Pts',(20.4893197886858,-17.7685114149095,-16.0151182561479));
#81427=CARTESIAN_POINT('Ctrl Pts',(20.4836041503097,-17.7600779795412,-16.0144631906337));
#81428=CARTESIAN_POINT('Ctrl Pts',(20.4774539859061,-17.7511429585327,-16.0137634472015));
#81429=CARTESIAN_POINT('Ctrl Pts',(20.4770797722772,-17.7505998408149,-16.0137208904825));
#81430=CARTESIAN_POINT('Ctrl Pts',(20.4637376061681,-17.7312549453425,-16.0122042912174));
#81431=CARTESIAN_POINT('Ctrl Pts',(20.4504667935286,-17.7126645454522,-16.0107197907439));
#81432=CARTESIAN_POINT('Ctrl Pts',(20.4097658136839,-17.6575566207473,-16.0062448339325));
#81433=CARTESIAN_POINT('Ctrl Pts',(20.3814524296277,-17.6217086687584,-16.0032337147627));
#81434=CARTESIAN_POINT('Ctrl Pts',(20.2814844878627,-17.5032285749942,-15.9929934745232));
#81435=CARTESIAN_POINT('Ctrl Pts',(20.2045911610316,-17.4252347967746,-15.9857628952117));
#81436=CARTESIAN_POINT('Ctrl Pts',(20.0804339718783,-17.317424623352,-15.9751939093095));
#81437=CARTESIAN_POINT('Ctrl Pts',(20.0374614036461,-17.2829552758222,-15.971707110043));
#81438=CARTESIAN_POINT('Ctrl Pts',(19.9656280004393,-17.2298045783962,-15.9661528278837));
#81439=CARTESIAN_POINT('Ctrl Pts',(19.9375729779295,-17.210082405946,-15.964046962912));
#81440=CARTESIAN_POINT('Ctrl Pts',(19.9000608369179,-17.1850512438452,-15.9613115242494));
#81441=CARTESIAN_POINT('Ctrl Pts',(19.891025843108,-17.1791218351412,-15.960658632483));
#81442=CARTESIAN_POINT('Ctrl Pts',(19.876150228919,-17.1695215480902,-15.9595932695886));
#81443=CARTESIAN_POINT('Ctrl Pts',(19.8703364509914,-17.1658096269315,-15.9591792697749));
#81444=CARTESIAN_POINT('Ctrl Pts',(19.8590454231097,-17.1586780859239,-15.9583797700264));
#81445=CARTESIAN_POINT('Ctrl Pts',(19.8535704726618,-17.1552549847753,-15.9579941439189));
#81446=CARTESIAN_POINT('Ctrl Pts',(19.8408898479375,-17.1474071478114,-15.9571056558735));
#81447=CARTESIAN_POINT('Ctrl Pts',(19.8336731231094,-17.1430004082056,-15.956603460327));
#81448=CARTESIAN_POINT('Ctrl Pts',(19.8141869539514,-17.131261292758,-15.955256591742));
#81449=CARTESIAN_POINT('Ctrl Pts',(19.8018692004384,-17.1240096605255,-15.9544148619002));
#81450=CARTESIAN_POINT('Ctrl Pts',(19.687971680864,-17.0585008012987,-15.9467174721327));
#81451=CARTESIAN_POINT('Ctrl Pts',(19.5817896987187,-17.0086371674994,-15.9401800340575));
#81452=CARTESIAN_POINT('Ctrl Pts',(19.3186486417966,-16.9107625227303,-15.9248116556554));
#81453=CARTESIAN_POINT('Ctrl Pts',(19.1592046897174,-16.8716987720604,-15.9161664053772));
#81454=CARTESIAN_POINT('Ctrl Pts',(18.9656472618229,-16.8474765239346,-15.90495304526));
#81455=CARTESIAN_POINT('Ctrl Pts',(18.9343369884688,-16.8442655841497,-15.9031159309338));
#81456=CARTESIAN_POINT('Ctrl Pts',(18.8958240926246,-16.8411818325507,-15.9008151250625));
#81457=CARTESIAN_POINT('Ctrl Pts',(18.8886767210276,-16.84064605487,-15.9003863995166));
#81458=CARTESIAN_POINT('Ctrl Pts',(18.8774430125444,-16.8398613062728,-15.8997096462996));
#81459=CARTESIAN_POINT('Ctrl Pts',(18.8733583627015,-16.839587870353,-15.899462969489));
#81460=CARTESIAN_POINT('Ctrl Pts',(18.8657059532007,-16.8390978920514,-15.8989996559279));
#81461=CARTESIAN_POINT('Ctrl Pts',(18.8621384295506,-16.8388785368364,-15.8987831786253));
#81462=CARTESIAN_POINT('Ctrl Pts',(18.8539725028342,-16.8383971961382,-15.8982865765393));
#81463=CARTESIAN_POINT('Ctrl Pts',(18.849373803297,-16.8381411829274,-15.8980061215519));
#81464=CARTESIAN_POINT('Ctrl Pts',(18.8351628063768,-16.8373965567705,-15.897137090127));
#81465=CARTESIAN_POINT('Ctrl Pts',(18.8255481414695,-16.8369584956144,-15.8965457938941));
#81466=CARTESIAN_POINT('Ctrl Pts',(18.7294004102483,-16.8332346462027,-15.8906016314718));
#81467=CARTESIAN_POINT('Ctrl Pts',(18.6427551493516,-16.835196115579,-15.8849957698359));
#81468=CARTESIAN_POINT('Ctrl Pts',(18.4300104430436,-16.8530983041842,-15.8709781186537));
#81469=CARTESIAN_POINT('Ctrl Pts',(18.3047396631587,-16.8750943410494,-15.8625167823198));
#81470=CARTESIAN_POINT('Ctrl Pts',(18.0889889624705,-16.9333445438758,-15.8480526013624));
#81471=CARTESIAN_POINT('Ctrl Pts',(17.9976063499515,-16.964856819913,-15.8419579293624));
#81472=CARTESIAN_POINT('Ctrl Pts',(17.8952172022191,-17.0082031399688,-15.8351790061739));
#81473=CARTESIAN_POINT('Ctrl Pts',(17.8818109212061,-17.0140431878553,-15.8342922471612));
#81474=CARTESIAN_POINT('Ctrl Pts',(17.8614116480839,-17.0231821446244,-15.8329439789958));
#81475=CARTESIAN_POINT('Ctrl Pts',(17.8543746313355,-17.0263811476855,-15.8324790654898));
#81476=CARTESIAN_POINT('Ctrl Pts',(17.8415803412243,-17.0322821571645,-15.8316340821913));
#81477=CARTESIAN_POINT('Ctrl Pts',(17.835817445277,-17.034971689508,-15.831253588536));
#81478=CARTESIAN_POINT('Ctrl Pts',(17.8233758132716,-17.0408465941867,-15.8304323316166));
#81479=CARTESIAN_POINT('Ctrl Pts',(17.8167014656041,-17.0440411034477,-15.8299918906153));
#81480=CARTESIAN_POINT('Ctrl Pts',(17.7985847175199,-17.0528292698749,-15.8287966171928));
#81481=CARTESIAN_POINT('Ctrl Pts',(17.7871757109439,-17.0584913548715,-15.8280441724757));
#81482=CARTESIAN_POINT('Ctrl Pts',(17.7311353448464,-17.0869363438208,-15.8243486684603));
#81483=CARTESIAN_POINT('Ctrl Pts',(17.6872694606958,-17.1111969910668,-15.8214579755489));
#81484=CARTESIAN_POINT('Ctrl Pts',(17.4954797331696,-17.2263440211844,-15.8087586060616));
#81485=CARTESIAN_POINT('Ctrl Pts',(17.3582177111238,-17.3336539369157,-15.7995651201117));
#81486=CARTESIAN_POINT('Ctrl Pts',(17.19129709884,-17.5009007949591,-15.7865788751071));
#81487=CARTESIAN_POINT('Ctrl Pts',(17.1489969915537,-17.5472276132431,-15.7830863866958));
#81488=CARTESIAN_POINT('Ctrl Pts',(17.0889996923105,-17.6191011162198,-15.7777011333854));
#81489=CARTESIAN_POINT('Ctrl Pts',(17.0697048262149,-17.6432728343305,-15.7758951095653));
#81490=CARTESIAN_POINT('Ctrl Pts',(17.0466234948629,-17.673524210655,-15.7736289380349));
#81491=CARTESIAN_POINT('Ctrl Pts',(17.0423282297889,-17.6792131236494,-15.7732025229752));
#81492=CARTESIAN_POINT('Ctrl Pts',(17.0356167548009,-17.6881962014242,-15.7725286096085));
#81493=CARTESIAN_POINT('Ctrl Pts',(17.0331811635645,-17.6914759130248,-15.7722824433926));
#81494=CARTESIAN_POINT('Ctrl Pts',(17.0286315565037,-17.6976395024459,-15.7718195518475));
#81495=CARTESIAN_POINT('Ctrl Pts',(17.0265153489583,-17.7005216934863,-15.77160298273));
#81496=CARTESIAN_POINT('Ctrl Pts',(17.0216819502259,-17.7071396722318,-15.7711054550512));
#81497=CARTESIAN_POINT('Ctrl Pts',(17.0189696857335,-17.7108789908125,-15.7708241616419));
#81498=CARTESIAN_POINT('Ctrl Pts',(17.0106032988427,-17.722493271639,-15.7699499942839));
#81499=CARTESIAN_POINT('Ctrl Pts',(17.004991109216,-17.7303980877424,-15.7693543548345));
#81500=CARTESIAN_POINT('Ctrl Pts',(16.9421416671983,-17.820222770141,-15.7625809764419));
#81501=CARTESIAN_POINT('Ctrl Pts',(16.8907261571511,-17.9060493411936,-15.7560680493768));
#81502=CARTESIAN_POINT('Ctrl Pts',(16.7684063382777,-18.1474645592063,-15.7382365648547));
#81503=CARTESIAN_POINT('Ctrl Pts',(16.7099350758424,-18.3085601099599,-15.7269007107454));
#81504=CARTESIAN_POINT('Ctrl Pts',(16.6614520670905,-18.5181762464437,-15.7134187920268));
#81505=CARTESIAN_POINT('Ctrl Pts',(16.6528139417587,-18.56171415668,-15.7106795622788));
#81506=CARTESIAN_POINT('Ctrl Pts',(16.6436144405759,-18.61716111556,-15.7072652715688));
#81507=CARTESIAN_POINT('Ctrl Pts',(16.6417764780847,-18.6288442963189,-15.7065499634193));
#81508=CARTESIAN_POINT('Ctrl Pts',(16.6389885125765,-18.6475880966758,-15.7054088041597));
#81509=CARTESIAN_POINT('Ctrl Pts',(16.6379760959988,-18.6546390491194,-15.7049809837439));
#81510=CARTESIAN_POINT('Ctrl Pts',(16.6361227657834,-18.6680264706376,-15.7041714091887));
#81511=CARTESIAN_POINT('Ctrl Pts',(16.635274926425,-18.6743618863432,-15.7037894401518));
#81512=CARTESIAN_POINT('Ctrl Pts',(16.6334140698792,-18.6887627946346,-15.7029237642299));
#81513=CARTESIAN_POINT('Ctrl Pts',(16.6324187836107,-18.696830507611,-15.7024406220194));
#81514=CARTESIAN_POINT('Ctrl Pts',(16.6299653959485,-18.7177062719833,-15.7011950717472));
#81515=CARTESIAN_POINT('Ctrl Pts',(16.6285777519007,-18.7305223843567,-15.7004348848485));
#81516=CARTESIAN_POINT('Ctrl Pts',(16.6203967177342,-18.8131247043734,-15.6955629085869));
#81517=CARTESIAN_POINT('Ctrl Pts',(16.6169563817282,-18.8832033388859,-15.6915582484701));
#81518=CARTESIAN_POINT('Ctrl Pts',(16.6171212268753,-19.1457165867496,-15.6768592614934));
#81519=CARTESIAN_POINT('Ctrl Pts',(16.6434647893585,-19.3371656425855,-15.6668249320135));
#81520=CARTESIAN_POINT('Ctrl Pts',(16.708705242865,-19.5703427336084,-15.6531662090734));
#81521=CARTESIAN_POINT('Ctrl Pts',(16.7238020963104,-19.6177853506364,-15.650302711385));
#81522=CARTESIAN_POINT('Ctrl Pts',(16.7421614448645,-19.669140807954,-15.6470652109916));
#81523=CARTESIAN_POINT('Ctrl Pts',(16.7437828787667,-19.673628420565,-15.6467811358882));
#81524=CARTESIAN_POINT('Ctrl Pts',(16.7454194499636,-19.6781104571738,-15.6464962048466));
#81525=CARTESIAN_POINT('Origin',(18.734,-18.952,0.));
#81526=CARTESIAN_POINT('',(16.7454194444943,-19.678110442195,-14.843838520965));
#81527=CARTESIAN_POINT('',(16.7486736625677,-19.6769293383554,-15.066381399119));
#81528=CARTESIAN_POINT('',(16.7454194499637,-19.6781104571739,0.));
#81529=CARTESIAN_POINT('',(16.6156459649053,-18.9502594248307,-15.110942953281));
#81530=CARTESIAN_POINT('Ctrl Pts',(16.7486736625677,-19.6769293383554,-15.066381399119));
#81531=CARTESIAN_POINT('Ctrl Pts',(16.6638907236804,-19.4439527091799,-15.0812352505063));
#81532=CARTESIAN_POINT('Ctrl Pts',(16.6178442275957,-19.196755842275,-15.0960891018936));
#81533=CARTESIAN_POINT('Ctrl Pts',(16.6156459649053,-18.9502594248307,-15.110942953281));
#81534=CARTESIAN_POINT('Ctrl Pts',(16.6170007608285,-18.9502051888479,-15.1101643145793));
#81535=CARTESIAN_POINT('Ctrl Pts',(16.6170691197414,-18.8695751089078,-15.1145731378411));
#81536=CARTESIAN_POINT('Ctrl Pts',(16.6217438741122,-18.7890199750102,-15.119036689108));
#81537=CARTESIAN_POINT('Ctrl Pts',(16.6337248049843,-18.6853612827869,-15.1250697269885));
#81538=CARTESIAN_POINT('Ctrl Pts',(16.6368453918934,-18.6618370352918,-15.1264584620397));
#81539=CARTESIAN_POINT('Ctrl Pts',(16.6412432750163,-18.632478810018,-15.1282217045135));
#81540=CARTESIAN_POINT('Ctrl Pts',(16.642150837834,-18.6265901327867,-15.1285768971463));
#81541=CARTESIAN_POINT('Ctrl Pts',(16.6437157802129,-18.6167132296185,-15.1291753239111));
#81542=CARTESIAN_POINT('Ctrl Pts',(16.6443597514526,-18.612722872974,-15.1294178270275));
#81543=CARTESIAN_POINT('Ctrl Pts',(16.6455594680531,-18.6054218501564,-15.1298629101726));
#81544=CARTESIAN_POINT('Ctrl Pts',(16.6461116697674,-18.6021106038405,-15.1300652910502));
#81545=CARTESIAN_POINT('Ctrl Pts',(16.6472681665263,-18.5952759684218,-15.1304841220257));
#81546=CARTESIAN_POINT('Ctrl Pts',(16.6478735058979,-18.5917528217064,-15.1307006328781));
#81547=CARTESIAN_POINT('Ctrl Pts',(16.6492800584961,-18.5836889554203,-15.1311975757814));
#81548=CARTESIAN_POINT('Ctrl Pts',(16.650087182348,-18.5791493227035,-15.131478339748));
#81549=CARTESIAN_POINT('Ctrl Pts',(16.6526294586288,-18.565116554505,-15.1323492617065));
#81550=CARTESIAN_POINT('Ctrl Pts',(16.654414669687,-18.5556327753986,-15.1329421562727));
#81551=CARTESIAN_POINT('Ctrl Pts',(16.6734315733765,-18.4582735619008,-15.1390706475135));
#81552=CARTESIAN_POINT('Ctrl Pts',(16.6961558783454,-18.3715728930258,-15.1448764856683));
#81553=CARTESIAN_POINT('Ctrl Pts',(16.7385997773342,-18.2433832521665,-15.1537504415924));
#81554=CARTESIAN_POINT('Ctrl Pts',(16.7542920791194,-18.2006570659467,-15.1567594586229));
#81555=CARTESIAN_POINT('Ctrl Pts',(16.78571002011,-18.1229505124147,-15.1622979063625));
#81556=CARTESIAN_POINT('Ctrl Pts',(16.8010330016433,-18.0878266598706,-15.1648270677989));
#81557=CARTESIAN_POINT('Ctrl Pts',(16.857652263453,-17.9670939618537,-15.1735859408722));
#81558=CARTESIAN_POINT('Ctrl Pts',(16.9037553332312,-17.8838573008273,-15.179735059823));
#81559=CARTESIAN_POINT('Ctrl Pts',(16.9803710678194,-17.7651504868338,-15.1886008576126));
#81560=CARTESIAN_POINT('Ctrl Pts',(17.0067075740656,-17.7271377223248,-15.1914572318686));
#81561=CARTESIAN_POINT('Ctrl Pts',(17.0414157516356,-17.6803902820937,-15.194994944838));
#81562=CARTESIAN_POINT('Ctrl Pts',(17.048643778364,-17.6708258791469,-15.1957201448677));
#81563=CARTESIAN_POINT('Ctrl Pts',(17.060317393222,-17.6556486655401,-15.1968733133754));
#81564=CARTESIAN_POINT('Ctrl Pts',(17.0647108064457,-17.6499962208848,-15.197303324918));
#81565=CARTESIAN_POINT('Ctrl Pts',(17.0730769213008,-17.6393445622146,-15.1981147191934));
#81566=CARTESIAN_POINT('Ctrl Pts',(17.0770437240328,-17.6343408359456,-15.1984963300181));
#81567=CARTESIAN_POINT('Ctrl Pts',(17.0860738322339,-17.6230555170312,-15.1993580737097));
#81568=CARTESIAN_POINT('Ctrl Pts',(17.091150549023,-17.6167847449192,-15.1998376618733));
#81569=CARTESIAN_POINT('Ctrl Pts',(17.1062386027625,-17.5983642777021,-15.2012488179835));
#81570=CARTESIAN_POINT('Ctrl Pts',(17.1163498928958,-17.5862968895233,-15.2021763319154));
#81571=CARTESIAN_POINT('Ctrl Pts',(17.2076539789396,-17.4797662679517,-15.2103951493466));
#81572=CARTESIAN_POINT('Ctrl Pts',(17.2969060023568,-17.3925221414867,-15.2173235739227));
#81573=CARTESIAN_POINT('Ctrl Pts',(17.5230012227813,-17.2075094013752,-15.2332790499738));
#81574=CARTESIAN_POINT('Ctrl Pts',(17.6647991631224,-17.1171813181652,-15.2421389788301));
#81575=CARTESIAN_POINT('Ctrl Pts',(17.8351421427705,-17.0351777594775,-15.2531371160311));
#81576=CARTESIAN_POINT('Ctrl Pts',(17.8546904645034,-17.0261319855951,-15.2544047265975));
#81577=CARTESIAN_POINT('Ctrl Pts',(17.8801226391083,-17.0148314362456,-15.256065187557));
#81578=CARTESIAN_POINT('Ctrl Pts',(17.8858840296342,-17.0123021136349,-15.2564420896998));
#81579=CARTESIAN_POINT('Ctrl Pts',(17.8947418675373,-17.0084604205186,-15.2570228209372));
#81580=CARTESIAN_POINT('Ctrl Pts',(17.8978303674907,-17.0071296559354,-15.2572255417991));
#81581=CARTESIAN_POINT('Ctrl Pts',(17.90420414822,-17.0044013270906,-15.257644409394));
#81582=CARTESIAN_POINT('Ctrl Pts',(17.907489768869,-17.0030047245972,-15.2578606137712));
#81583=CARTESIAN_POINT('Ctrl Pts',(17.9149824864291,-16.9998421860427,-15.2583542929644));
#81584=CARTESIAN_POINT('Ctrl Pts',(17.9191917530114,-16.9980815426766,-15.2586320832073));
#81585=CARTESIAN_POINT('Ctrl Pts',(17.9301572903825,-16.9935364954571,-15.259356860997));
#81586=CARTESIAN_POINT('Ctrl Pts',(17.9369222789644,-16.9907734696079,-15.259805090379));
#81587=CARTESIAN_POINT('Ctrl Pts',(17.9802234226111,-16.9733490141404,-15.2626804287361));
#81588=CARTESIAN_POINT('Ctrl Pts',(18.0171457755562,-16.9596751222136,-15.2651607773159));
#81589=CARTESIAN_POINT('Ctrl Pts',(18.235201716319,-16.8857657503663,-15.2798884079933));
#81590=CARTESIAN_POINT('Ctrl Pts',(18.4234383087793,-16.849219367164,-15.2928183246153));
#81591=CARTESIAN_POINT('Ctrl Pts',(18.6690529453782,-16.8352791692237,-15.3086312183993));
#81592=CARTESIAN_POINT('Ctrl Pts',(18.7241703607051,-16.8343056418313,-15.3121204590878));
#81593=CARTESIAN_POINT('Ctrl Pts',(18.8135629070257,-16.8362175210011,-15.3176781746887));
#81594=CARTESIAN_POINT('Ctrl Pts',(18.8478374835046,-16.8377845430761,-15.3197850908614));
#81595=CARTESIAN_POINT('Ctrl Pts',(18.8928425358842,-16.8409398699132,-15.3225216745292));
#81596=CARTESIAN_POINT('Ctrl Pts',(18.903618791606,-16.8417783774286,-15.3231746845181));
#81597=CARTESIAN_POINT('Ctrl Pts',(18.9212612533888,-16.8432871684874,-15.3242401909176));
#81598=CARTESIAN_POINT('Ctrl Pts',(18.9281313432878,-16.8439085394338,-15.3246542168083));
#81599=CARTESIAN_POINT('Ctrl Pts',(18.9414258997368,-16.8451765177197,-15.3254537327886));
#81600=CARTESIAN_POINT('Ctrl Pts',(18.9478506781229,-16.8458189588116,-15.3258393492298));
#81601=CARTESIAN_POINT('Ctrl Pts',(18.9626811672482,-16.8473704830161,-15.326727766235));
#81602=CARTESIAN_POINT('Ctrl Pts',(18.9710846082253,-16.8483005510008,-15.3272299007503));
#81603=CARTESIAN_POINT('Ctrl Pts',(18.9936755513015,-16.8509379350574,-15.3285764974201));
#81604=CARTESIAN_POINT('Ctrl Pts',(19.0078518662731,-16.8527386149092,-15.3294180182596));
#81605=CARTESIAN_POINT('Ctrl Pts',(19.1377451283051,-16.8705758994455,-15.3370990129157));
#81606=CARTESIAN_POINT('Ctrl Pts',(19.2519741142662,-16.8960222535672,-15.3436218860048));
#81607=CARTESIAN_POINT('Ctrl Pts',(19.5189116212569,-16.9791626350241,-15.3589277184868));
#81608=CARTESIAN_POINT('Ctrl Pts',(19.668172525631,-17.0453056453673,-15.3675276002886));
#81609=CARTESIAN_POINT('Ctrl Pts',(19.8363822074808,-17.1443773754407,-15.3787365995727));
#81610=CARTESIAN_POINT('Ctrl Pts',(19.8640114923998,-17.1615196594594,-15.3806328928087));
#81611=CARTESIAN_POINT('Ctrl Pts',(19.8972958414608,-17.1832478405104,-15.3829995676429));
#81612=CARTESIAN_POINT('Ctrl Pts',(19.9033378842848,-17.1872364675708,-15.3834325726173));
#81613=CARTESIAN_POINT('Ctrl Pts',(19.9127774099826,-17.1935376865304,-15.3841145845471));
#81614=CARTESIAN_POINT('Ctrl Pts',(19.9161888857246,-17.1958293568144,-15.384362205581));
#81615=CARTESIAN_POINT('Ctrl Pts',(19.9225528715413,-17.2001313318991,-15.3848263111737));
#81616=CARTESIAN_POINT('Ctrl Pts',(19.9255069742107,-17.2021391802564,-15.3850426303395));
#81617=CARTESIAN_POINT('Ctrl Pts',(19.9322384985863,-17.2067394206386,-15.3855375738613));
#81618=CARTESIAN_POINT('Ctrl Pts',(19.9360125820067,-17.2093365955661,-15.3858165200582));
#81619=CARTESIAN_POINT('Ctrl Pts',(19.9475864351039,-17.2173567484563,-15.3866763526846));
#81620=CARTESIAN_POINT('Ctrl Pts',(19.9553580313984,-17.2228199061397,-15.3872598780031));
#81621=CARTESIAN_POINT('Ctrl Pts',(20.0609994710828,-17.2981495661774,-15.3952735575706));
#81622=CARTESIAN_POINT('Ctrl Pts',(20.1527691273615,-17.376171226247,-15.4031857664361));
#81623=CARTESIAN_POINT('Ctrl Pts',(20.3139826238442,-17.5387862437774,-15.4183136523095));
#81624=CARTESIAN_POINT('Ctrl Pts',(20.3844953901134,-17.6218170573477,-15.4255015744608));
#81625=CARTESIAN_POINT('Ctrl Pts',(20.4921552110227,-17.7704071972237,-15.4372889045334));
#81626=CARTESIAN_POINT('Ctrl Pts',(20.5327621513991,-17.833193430292,-15.4419888857415));
#81627=CARTESIAN_POINT('Ctrl Pts',(20.5793099886945,-17.914275495576,-15.4477160602456));
#81628=CARTESIAN_POINT('Ctrl Pts',(20.5884357176153,-17.9306727721841,-15.4488577274203));
#81629=CARTESIAN_POINT('Ctrl Pts',(20.6013989038248,-17.9547119902182,-15.4505080075677));
#81630=CARTESIAN_POINT('Ctrl Pts',(20.605409799819,-17.9622589202485,-15.4510227831713));
#81631=CARTESIAN_POINT('Ctrl Pts',(20.6123664339373,-17.9755420560458,-15.4519230902177));
#81632=CARTESIAN_POINT('Ctrl Pts',(20.6153318504578,-17.9812677782554,-15.4523093148902));
#81633=CARTESIAN_POINT('Ctrl Pts',(20.6210425004237,-17.9924185458965,-15.4530579237651));
#81634=CARTESIAN_POINT('Ctrl Pts',(20.6237906108457,-17.9978420393821,-15.4534204064972));
#81635=CARTESIAN_POINT('Ctrl Pts',(20.6303094713962,-18.0108458856296,-15.4542856898601));
#81636=CARTESIAN_POINT('Ctrl Pts',(20.6340582067159,-18.0184372048122,-15.4547877172227));
#81637=CARTESIAN_POINT('Ctrl Pts',(20.6474512464169,-18.045973438777,-15.4565977314761));
#81638=CARTESIAN_POINT('Ctrl Pts',(20.6568280796822,-18.0660473868922,-15.4578964409773));
#81639=CARTESIAN_POINT('Ctrl Pts',(20.741595176437,-18.2552053197196,-15.469951458362));
#81640=CARTESIAN_POINT('Ctrl Pts',(20.7948152000208,-18.4333402024837,-15.4798561845685));
#81641=CARTESIAN_POINT('Ctrl Pts',(20.8369504128257,-18.6955635533118,-15.4943330380546));
#81642=CARTESIAN_POINT('Ctrl Pts',(20.845174292267,-18.7756447490726,-15.4987559730682));
#81643=CARTESIAN_POINT('Ctrl Pts',(20.8504595433111,-18.8920665410086,-15.5054217007623));
#81644=CARTESIAN_POINT('Ctrl Pts',(20.8511738231199,-18.9281741761837,-15.5075220242888));
#81645=CARTESIAN_POINT('Ctrl Pts',(20.8509210469528,-18.9717509256829,-15.5101153368248));
#81646=CARTESIAN_POINT('Ctrl Pts',(20.8508381614858,-18.9792215429347,-15.5105620006315));
#81647=CARTESIAN_POINT('Ctrl Pts',(20.8506475586361,-18.990851272713,-15.5112607848848));
#81648=CARTESIAN_POINT('Ctrl Pts',(20.8505671202302,-18.9950108561649,-15.5115114049122));
#81649=CARTESIAN_POINT('Ctrl Pts',(20.850394970169,-19.0027350487422,-15.5119781176861));
#81650=CARTESIAN_POINT('Ctrl Pts',(20.8503065136778,-19.0062996729991,-15.5121940264597));
#81651=CARTESIAN_POINT('Ctrl Pts',(20.850085804409,-19.0143714707114,-15.5126841203791));
#81652=CARTESIAN_POINT('Ctrl Pts',(20.8499481577756,-19.0188784323672,-15.5129586025568));
#81653=CARTESIAN_POINT('Ctrl Pts',(20.849498006687,-19.0322205860429,-15.5137735637074));
#81654=CARTESIAN_POINT('Ctrl Pts',(20.8491445593857,-19.0410541709702,-15.5143162499787));
#81655=CARTESIAN_POINT('Ctrl Pts',(20.8461241401415,-19.1063081108626,-15.5183468313878));
#81656=CARTESIAN_POINT('Ctrl Pts',(20.8412556260364,-19.1625989035414,-15.5219434801864));
#81657=CARTESIAN_POINT('Ctrl Pts',(20.8131046449385,-19.3843401555385,-15.5364180765149));
#81658=CARTESIAN_POINT('Ctrl Pts',(20.7725261295108,-19.5469898889839,-15.5476594745444));
#81659=CARTESIAN_POINT('Ctrl Pts',(20.6924878529298,-19.7578757422094,-15.5621968538009));
#81660=CARTESIAN_POINT('Ctrl Pts',(20.66947368846,-19.811681890864,-15.5659093240687));
#81661=CARTESIAN_POINT('Ctrl Pts',(20.6288206965622,-19.8967890768006,-15.5717793660662));
#81662=CARTESIAN_POINT('Ctrl Pts',(20.6125643597269,-19.9287128872708,-15.5739809831105));
#81663=CARTESIAN_POINT('Ctrl Pts',(20.5902763260031,-19.9698643021249,-15.5768204393296));
#81664=CARTESIAN_POINT('Ctrl Pts',(20.5849725914846,-19.979477497907,-15.5774838714361));
#81665=CARTESIAN_POINT('Ctrl Pts',(20.5761967548112,-19.9950954979423,-15.5785620280071));
#81666=CARTESIAN_POINT('Ctrl Pts',(20.5727695531084,-20.0011251753757,-15.5789783526019));
#81667=CARTESIAN_POINT('Ctrl Pts',(20.5661017523705,-20.0127231845394,-15.5797793415378));
#81668=CARTESIAN_POINT('Ctrl Pts',(20.5628652492898,-20.018293771254,-15.5801641478218));
#81669=CARTESIAN_POINT('Ctrl Pts',(20.5553678073458,-20.0310636185869,-15.5810465119199));
#81670=CARTESIAN_POINT('Ctrl Pts',(20.5510895060822,-20.038252600708,-15.5815434328393));
#81671=CARTESIAN_POINT('Ctrl Pts',(20.5395461984696,-20.0573901879183,-15.5828668838649));
#81672=CARTESIAN_POINT('Ctrl Pts',(20.5322051523821,-20.0692926144422,-15.5836906305744));
#81673=CARTESIAN_POINT('Ctrl Pts',(20.4711016089967,-20.1662006504558,-15.5904048556163));
#81674=CARTESIAN_POINT('Ctrl Pts',(20.4114583636735,-20.247354159216,-15.5960656517049));
#81675=CARTESIAN_POINT('Ctrl Pts',(20.2351968897145,-20.4544873169829,-15.6110491234602));
#81676=CARTESIAN_POINT('Ctrl Pts',(20.108705877371,-20.5710220549652,-15.6200588730909));
#81677=CARTESIAN_POINT('Ctrl Pts',(19.937182119321,-20.6943067283641,-15.6320939663138));
#81678=CARTESIAN_POINT('Ctrl Pts',(19.9041445611221,-20.716664611552,-15.6344072888017));
#81679=CARTESIAN_POINT('Ctrl Pts',(19.8640134933786,-20.7422004286718,-15.6372366759696));
#81680=CARTESIAN_POINT('Ctrl Pts',(19.8575068967892,-20.7462910351449,-15.6376960082582));
#81681=CARTESIAN_POINT('Ctrl Pts',(19.8474045632327,-20.7525657380572,-15.6384103297905));
#81682=CARTESIAN_POINT('Ctrl Pts',(19.8438242700708,-20.7547747467025,-15.6386637088752));
#81683=CARTESIAN_POINT('Ctrl Pts',(19.8372005148472,-20.7588343342487,-15.6391329295904));
#81684=CARTESIAN_POINT('Ctrl Pts',(19.8341589573712,-20.760687909878,-15.6393485705007));
#81685=CARTESIAN_POINT('Ctrl Pts',(19.8273078768079,-20.7648393969629,-15.6398347007006));
#81686=CARTESIAN_POINT('Ctrl Pts',(19.8234958046325,-20.7671329657969,-15.640105466264));
#81687=CARTESIAN_POINT('Ctrl Pts',(19.813723307694,-20.7729708036188,-15.6408002325388));
#81688=CARTESIAN_POINT('Ctrl Pts',(19.8077526993204,-20.7764978011684,-15.6412253146944));
#81689=CARTESIAN_POINT('Ctrl Pts',(19.7727732468777,-20.7969299286036,-15.6437187512228));
#81690=CARTESIAN_POINT('Ctrl Pts',(19.7433845866367,-20.8131713419148,-15.6458258031895));
#81691=CARTESIAN_POINT('Ctrl Pts',(19.6974370899012,-20.8371555347414,-15.649124335273));
#81692=CARTESIAN_POINT('Ctrl Pts',(19.6811417857406,-20.8453950506753,-15.650294980898));
#81693=CARTESIAN_POINT('Ctrl Pts',(19.6425587959565,-20.8642813444969,-15.6530654005765));
#81694=CARTESIAN_POINT('Ctrl Pts',(19.6201874491395,-20.8747508327259,-15.6546706931166));
#81695=CARTESIAN_POINT('Ctrl Pts',(19.5566267091408,-20.9031514793808,-15.659219545964));
#81696=CARTESIAN_POINT('Ctrl Pts',(19.5150427438893,-20.9201663677265,-15.6621813381257));
#81697=CARTESIAN_POINT('Ctrl Pts',(19.3704830766048,-20.97401249267,-15.6723715694895));
#81698=CARTESIAN_POINT('Ctrl Pts',(19.2652050146525,-21.0041866207842,-15.6796016017227));
#81699=CARTESIAN_POINT('Ctrl Pts',(19.1041215629254,-21.0371211305131,-15.6901694386007));
#81700=CARTESIAN_POINT('Ctrl Pts',(19.0497690453268,-21.0460417449079,-15.6936556397206));
#81701=CARTESIAN_POINT('Ctrl Pts',(18.9611055328422,-21.0570623259829,-15.6992090807324));
#81702=CARTESIAN_POINT('Ctrl Pts',(18.9269852576525,-21.0604641864612,-15.7013146882049));
#81703=CARTESIAN_POINT('Ctrl Pts',(18.8820200993857,-21.0638465432519,-15.7040498464714));
#81704=CARTESIAN_POINT('Ctrl Pts',(18.8712382291001,-21.0645746015991,-15.7047027093586));
#81705=CARTESIAN_POINT('Ctrl Pts',(18.8535659120658,-21.0656320796666,-15.7057680372571));
#81706=CARTESIAN_POINT('Ctrl Pts',(18.8466786915673,-21.0660104280117,-15.7061820307599));
#81707=CARTESIAN_POINT('Ctrl Pts',(18.8333408041358,-21.0666777761061,-15.7069815267012));
#81708=CARTESIAN_POINT('Ctrl Pts',(18.8268904305926,-21.0669709363141,-15.7073671552684));
#81709=CARTESIAN_POINT('Ctrl Pts',(18.8119899272544,-21.0675798432687,-15.7082556609591));
#81710=CARTESIAN_POINT('Ctrl Pts',(18.8035390090154,-21.0678744838453,-15.7087578716069));
#81711=CARTESIAN_POINT('Ctrl Pts',(18.7807983235475,-21.0685309442126,-15.7101048072834));
#81712=CARTESIAN_POINT('Ctrl Pts',(18.7665061264124,-21.0687986884836,-15.710946588652));
#81713=CARTESIAN_POINT('Ctrl Pts',(18.6350479192716,-21.069929634011,-15.7186480889499));
#81714=CARTESIAN_POINT('Ctrl Pts',(18.5179952260785,-21.0612094921747,-15.7251891787752));
#81715=CARTESIAN_POINT('Ctrl Pts',(18.2404051985606,-21.0171651317415,-15.7405741040444));
#81716=CARTESIAN_POINT('Ctrl Pts',(18.0821079303989,-20.972783815009,-15.7492315240695));
#81717=CARTESIAN_POINT('Ctrl Pts',(17.9016682142281,-20.8987629912337,-15.7604463261497));
#81718=CARTESIAN_POINT('Ctrl Pts',(17.873071016026,-20.8862862759913,-15.7622678426905));
#81719=CARTESIAN_POINT('Ctrl Pts',(17.8382748875729,-20.870180548458,-15.7645512755516));
#81720=CARTESIAN_POINT('Ctrl Pts',(17.8318034371261,-20.8671452822531,-15.7649788474803));
#81721=CARTESIAN_POINT('Ctrl Pts',(17.8216539277324,-20.862322058866,-15.7656541828522));
#81722=CARTESIAN_POINT('Ctrl Pts',(17.8179653976249,-20.8605560853097,-15.7659006048208));
#81723=CARTESIAN_POINT('Ctrl Pts',(17.811062020589,-20.8572263033511,-15.7663637072348));
#81724=CARTESIAN_POINT('Ctrl Pts',(17.8078460100684,-20.8556650354194,-15.766580229846));
#81725=CARTESIAN_POINT('Ctrl Pts',(17.8004896175149,-20.8520706939302,-15.7670772915019));
#81726=CARTESIAN_POINT('Ctrl Pts',(17.7963519275842,-20.8500322356339,-15.7673581630583));
#81727=CARTESIAN_POINT('Ctrl Pts',(17.7855281762086,-20.844655817947,-15.7680962215253));
#81728=CARTESIAN_POINT('Ctrl Pts',(17.7788531372778,-20.8412959833172,-15.7685547244682));
#81729=CARTESIAN_POINT('Ctrl Pts',(17.734172197797,-20.8185088372921,-15.7716455918281));
#81730=CARTESIAN_POINT('Ctrl Pts',(17.6967462941565,-20.7979726583724,-15.7743405541364));
#81731=CARTESIAN_POINT('Ctrl Pts',(17.6537625704002,-20.7726669046396,-15.7775396716289));
#81732=CARTESIAN_POINT('Ctrl Pts',(17.6475742249394,-20.7689809892071,-15.7780028293955));
#81733=CARTESIAN_POINT('Ctrl Pts',(17.5067332157273,-20.6841162183012,-15.7886010738821));
#81734=CARTESIAN_POINT('Ctrl Pts',(17.3815204063515,-20.5882189996179,-15.7991743274516));
#81735=CARTESIAN_POINT('Ctrl Pts',(17.1996368762811,-20.4136489959253,-15.8155534556939));
#81736=CARTESIAN_POINT('Ctrl Pts',(17.1356824252017,-20.3434284383633,-15.8215790815982));
#81737=CARTESIAN_POINT('Ctrl Pts',(17.0633767559959,-20.2524468135082,-15.8287171598595));
#81738=CARTESIAN_POINT('Ctrl Pts',(17.0503589583529,-20.2355485317303,-15.830017206774));
#81739=CARTESIAN_POINT('Ctrl Pts',(17.0322147374942,-20.2112445779466,-15.8318514329844));
#81740=CARTESIAN_POINT('Ctrl Pts',(17.0268770680754,-20.2039989161242,-15.8323938663043));
#81741=CARTESIAN_POINT('Ctrl Pts',(17.0177495690668,-20.1914418205486,-15.8333264533301));
#81742=CARTESIAN_POINT('Ctrl Pts',(17.0139378247976,-20.1861465403754,-15.8337174542962));
#81743=CARTESIAN_POINT('Ctrl Pts',(17.0066870490848,-20.1759749071547,-15.8344642324701));
#81744=CARTESIAN_POINT('Ctrl Pts',(17.00324404074,-20.1711014782833,-15.8348201605029));
#81745=CARTESIAN_POINT('Ctrl Pts',(16.9943461598524,-20.1583932419596,-15.8357434985385));
#81746=CARTESIAN_POINT('Ctrl Pts',(16.9889235584248,-20.1505359216073,-15.8363096724455));
#81747=CARTESIAN_POINT('Ctrl Pts',(16.9706219367321,-20.1236294342209,-15.8382327302425));
#81748=CARTESIAN_POINT('Ctrl Pts',(16.957999916433,-20.1044068245473,-15.8395799220599));
#81749=CARTESIAN_POINT('Ctrl Pts',(16.8645247607842,-19.9568649544033,-15.8497291340341));
#81750=CARTESIAN_POINT('Ctrl Pts',(16.7973961928405,-19.8204578628901,-15.857987038895));
#81751=CARTESIAN_POINT('Ctrl Pts',(16.7454194501833,-19.6781104577752,-15.8662164286365));
#81752=CARTESIAN_POINT('',(16.6170002518852,-18.9530327061848,-14.8907771671312));
#81753=CARTESIAN_POINT('Ctrl Pts',(16.7454194499636,-19.6781104571738,-15.6464962048466));
#81754=CARTESIAN_POINT('Ctrl Pts',(16.7464618210687,-19.6809651728509,-15.646314725492));
#81755=CARTESIAN_POINT('Ctrl Pts',(16.7475103329493,-19.6838176265005,-15.6461328989071));
#81756=CARTESIAN_POINT('Ctrl Pts',(16.7501831766152,-19.6910409693967,-15.6456711856327));
#81757=CARTESIAN_POINT('Ctrl Pts',(16.7518158016566,-19.6954087341947,-15.6453908199843));
#81758=CARTESIAN_POINT('Ctrl Pts',(16.7547310336525,-19.7031299819739,-15.6448930447428));
#81759=CARTESIAN_POINT('Ctrl Pts',(16.756007757495,-19.7064856389605,-15.6446759886965));
#81760=CARTESIAN_POINT('Ctrl Pts',(16.7587298590321,-19.7135858325257,-15.6442151686796));
#81761=CARTESIAN_POINT('Ctrl Pts',(16.7601773285189,-19.717329452609,-15.6439712857206));
#81762=CARTESIAN_POINT('Ctrl Pts',(16.764107895231,-19.7274098375799,-15.6433121671797));
#81763=CARTESIAN_POINT('Ctrl Pts',(16.7666108941802,-19.7337387185235,-15.6428957624867));
#81764=CARTESIAN_POINT('Ctrl Pts',(16.7791207397704,-19.7649294743618,-15.6408312027123));
#81765=CARTESIAN_POINT('Ctrl Pts',(16.7895680676519,-19.7896106239208,-15.6391585752494));
#81766=CARTESIAN_POINT('Ctrl Pts',(16.8210382187307,-19.860193131573,-15.6342757155358));
#81767=CARTESIAN_POINT('Ctrl Pts',(16.8432373327428,-19.9055477946504,-15.6310148770947));
#81768=CARTESIAN_POINT('Ctrl Pts',(16.9295816576105,-20.0670626117623,-15.619052347282));
#81769=CARTESIAN_POINT('Ctrl Pts',(17.0029892562356,-20.1779261337073,-15.6101841445996));
#81770=CARTESIAN_POINT('Ctrl Pts',(17.1511162416845,-20.3615483824414,-15.5948582182858));
#81771=CARTESIAN_POINT('Ctrl Pts',(17.2217357575043,-20.4370622810837,-15.5883172728628));
#81772=CARTESIAN_POINT('Ctrl Pts',(17.307910783786,-20.5166583496608,-15.581156619092));
#81773=CARTESIAN_POINT('Ctrl Pts',(17.318321337597,-20.5260839061179,-15.5803038107971));
#81774=CARTESIAN_POINT('Ctrl Pts',(17.3350950535345,-20.5409695475882,-15.5789489182868));
#81775=CARTESIAN_POINT('Ctrl Pts',(17.341398060896,-20.5464965082337,-15.578444033336));
#81776=CARTESIAN_POINT('Ctrl Pts',(17.3526049390228,-20.5562064162179,-15.5775537326945));
#81777=CARTESIAN_POINT('Ctrl Pts',(17.3574953646269,-20.5604046538568,-15.5771676843011));
#81778=CARTESIAN_POINT('Ctrl Pts',(17.367682196607,-20.5690691566743,-15.5763685822068));
#81779=CARTESIAN_POINT('Ctrl Pts',(17.3729815138332,-20.5735318928106,-15.5759556763934));
#81780=CARTESIAN_POINT('Ctrl Pts',(17.3867089328402,-20.5849775168373,-15.5748932001708));
#81781=CARTESIAN_POINT('Ctrl Pts',(17.395169517965,-20.5919212594894,-15.5742452275677));
#81782=CARTESIAN_POINT('Ctrl Pts',(17.431306814496,-20.6211136683047,-15.5715060245732));
#81783=CARTESIAN_POINT('Ctrl Pts',(17.459488095506,-20.6427304917977,-15.5694401327033));
#81784=CARTESIAN_POINT('Ctrl Pts',(17.534931611253,-20.6976415973162,-15.5640773286126));
#81785=CARTESIAN_POINT('Ctrl Pts',(17.5830375216308,-20.7297276755951,-15.5608243468964));
#81786=CARTESIAN_POINT('Ctrl Pts',(17.7707930760212,-20.8441379628006,-15.5486248535451));
#81787=CARTESIAN_POINT('Ctrl Pts',(17.9184014546629,-20.9122926399963,-15.5400738392206));
#81788=CARTESIAN_POINT('Ctrl Pts',(18.0929192853502,-20.9697151258336,-15.5298130920824));
#81789=CARTESIAN_POINT('Ctrl Pts',(18.1136108022514,-20.9761729184677,-15.5285935048515));
#81790=CARTESIAN_POINT('Ctrl Pts',(18.1746751932879,-20.9942067886059,-15.5249758342402));
#81791=CARTESIAN_POINT('Ctrl Pts',(18.21529521678,-21.0048998087632,-15.5225459165641));
#81792=CARTESIAN_POINT('Ctrl Pts',(18.2634485539831,-21.0160556315644,-15.5196092817676));
#81793=CARTESIAN_POINT('Ctrl Pts',(18.2707026383087,-21.0176959758177,-15.5191654058786));
#81794=CARTESIAN_POINT('Ctrl Pts',(18.2824589206213,-21.0202893489095,-15.5184434191252));
#81795=CARTESIAN_POINT('Ctrl Pts',(18.286955918693,-21.0212659968284,-15.5181666261419));
#81796=CARTESIAN_POINT('Ctrl Pts',(18.29495096904,-21.0229750653415,-15.5176733684641));
#81797=CARTESIAN_POINT('Ctrl Pts',(18.2984477280889,-21.0237132984725,-15.5174572398138));
#81798=CARTESIAN_POINT('Ctrl Pts',(18.3059565595425,-21.025278706175,-15.516992268415));
#81799=CARTESIAN_POINT('Ctrl Pts',(18.3099691085308,-21.0261030791211,-15.5167432751951));
#81800=CARTESIAN_POINT('Ctrl Pts',(18.3210204078847,-21.0283401447055,-15.5160561112889));
#81801=CARTESIAN_POINT('Ctrl Pts',(18.3280639146646,-21.0297286712271,-15.5156165988955));
#81802=CARTESIAN_POINT('Ctrl Pts',(18.3661847034743,-21.0370424015846,-15.5132300037682));
#81803=CARTESIAN_POINT('Ctrl Pts',(18.3973830193666,-21.0423058791424,-15.5112485906621));
#81804=CARTESIAN_POINT('Ctrl Pts',(18.5904483669883,-21.0704439978995,-15.4988614468198));
#81805=CARTESIAN_POINT('Ctrl Pts',(18.7543926853166,-21.0752041806364,-15.4878510943337));
#81806=CARTESIAN_POINT('Ctrl Pts',(19.0338618070423,-21.0509218147031,-15.4695259693753));
#81807=CARTESIAN_POINT('Ctrl Pts',(19.1494464943902,-21.0311349041748,-15.4620691876712));
#81808=CARTESIAN_POINT('Ctrl Pts',(19.2766584371441,-20.9983174473749,-15.4540472948938));
#81809=CARTESIAN_POINT('Ctrl Pts',(19.2904615647938,-20.994607112851,-15.453179126206));
#81810=CARTESIAN_POINT('Ctrl Pts',(19.3123692430935,-20.9884796863122,-15.4518045712465));
#81811=CARTESIAN_POINT('Ctrl Pts',(19.3204985289586,-20.9861533798828,-15.4512952552727));
#81812=CARTESIAN_POINT('Ctrl Pts',(19.3348106924406,-20.9819648280142,-15.4503998127639));
#81813=CARTESIAN_POINT('Ctrl Pts',(19.3409993553586,-20.9801228944896,-15.4500130298047));
#81814=CARTESIAN_POINT('Ctrl Pts',(19.3537815600591,-20.976254775446,-15.4492149734379));
#81815=CARTESIAN_POINT('Ctrl Pts',(19.3603738273923,-20.9742246186303,-15.4488038352554));
#81816=CARTESIAN_POINT('Ctrl Pts',(19.3772687434226,-20.9689311129403,-15.4477512460136));
#81817=CARTESIAN_POINT('Ctrl Pts',(19.3875566197258,-20.965621002567,-15.4471113355632));
#81818=CARTESIAN_POINT('Ctrl Pts',(19.430379956665,-20.9514798810135,-15.4444516256623));
#81819=CARTESIAN_POINT('Ctrl Pts',(19.462676266121,-20.9399376082191,-15.4424553333884));
#81820=CARTESIAN_POINT('Ctrl Pts',(19.5460739492627,-20.9078266536128,-15.4373138949028));
#81821=CARTESIAN_POINT('Ctrl Pts',(19.5966791399523,-20.8860391267957,-15.434208084708));
#81822=CARTESIAN_POINT('Ctrl Pts',(19.7450257999569,-20.8151872147673,-15.4250667253287));
#81823=CARTESIAN_POINT('Ctrl Pts',(19.8398767713543,-20.7605013737198,-15.4191799156477));
#81824=CARTESIAN_POINT('Ctrl Pts',(19.9655431323308,-20.6744511242105,-15.4108879478435));
#81825=CARTESIAN_POINT('Ctrl Pts',(20.0002580291228,-20.649093626091,-15.4085384512978));
#81826=CARTESIAN_POINT('Ctrl Pts',(20.0938029621756,-20.5762947740697,-15.4019765739369));
#81827=CARTESIAN_POINT('Ctrl Pts',(20.1508964488008,-20.5267379112893,-15.3977073727041));
#81828=CARTESIAN_POINT('Ctrl Pts',(20.2120392649715,-20.467644767645,-15.3926678153139));
#81829=CARTESIAN_POINT('Ctrl Pts',(20.2188211745769,-20.4610013924521,-15.3921019241724));
#81830=CARTESIAN_POINT('Ctrl Pts',(20.2288083491485,-20.4510857139536,-15.3912578532898));
#81831=CARTESIAN_POINT('Ctrl Pts',(20.2320481543938,-20.4478481556217,-15.3909823437547));
#81832=CARTESIAN_POINT('Ctrl Pts',(20.2377957075304,-20.4420671890166,-15.3904904932399));
#81833=CARTESIAN_POINT('Ctrl Pts',(20.2403075502035,-20.4395279230118,-15.390274481031));
#81834=CARTESIAN_POINT('Ctrl Pts',(20.2456963630598,-20.4340526315139,-15.3898087557144));
#81835=CARTESIAN_POINT('Ctrl Pts',(20.2485711696053,-20.4311146230777,-15.389558886848));
#81836=CARTESIAN_POINT('Ctrl Pts',(20.2564882208778,-20.4229762356269,-15.3888668906742));
#81837=CARTESIAN_POINT('Ctrl Pts',(20.2615123043431,-20.4177583788191,-15.3884233908925));
#81838=CARTESIAN_POINT('Ctrl Pts',(20.2889763028575,-20.3889405723166,-15.3859754209218));
#81839=CARTESIAN_POINT('Ctrl Pts',(20.3108948352396,-20.3648524054532,-15.3839345442539));
#81840=CARTESIAN_POINT('Ctrl Pts',(20.4389281076429,-20.2174539255712,-15.3715279130892));
#81841=CARTESIAN_POINT('Ctrl Pts',(20.5310941521381,-20.0827546295301,-15.3605727186579));
#81842=CARTESIAN_POINT('Ctrl Pts',(20.6613730510475,-19.8354957893216,-15.3423172744141));
#81843=CARTESIAN_POINT('Ctrl Pts',(20.7071813389951,-19.7278188547983,-15.334877080425));
#81844=CARTESIAN_POINT('Ctrl Pts',(20.7483642047674,-19.603329434519,-15.3268706247309));
#81845=CARTESIAN_POINT('Ctrl Pts',(20.7527146989843,-19.5897179325849,-15.3260026566042));
#81846=CARTESIAN_POINT('Ctrl Pts',(20.7594193959784,-19.5679843736217,-15.3246283581713));
#81847=CARTESIAN_POINT('Ctrl Pts',(20.7618632717442,-19.5598906418935,-15.3241190998638));
#81848=CARTESIAN_POINT('Ctrl Pts',(20.7660879209208,-19.5455902381051,-15.3232237244325));
#81849=CARTESIAN_POINT('Ctrl Pts',(20.7678888954473,-19.5393896930787,-15.3228369511937));
#81850=CARTESIAN_POINT('Ctrl Pts',(20.7715552206011,-19.5265479147972,-15.3220388820318));
#81851=CARTESIAN_POINT('Ctrl Pts',(20.7734165371927,-19.5199056021499,-15.3216277214958));
#81852=CARTESIAN_POINT('Ctrl Pts',(20.7781109544491,-19.5028323104883,-15.3205750070277));
#81853=CARTESIAN_POINT('Ctrl Pts',(20.7808967178448,-19.4923884356752,-15.3199349944245));
#81854=CARTESIAN_POINT('Ctrl Pts',(20.7921897536862,-19.4487099953196,-15.3172742918244));
#81855=CARTESIAN_POINT('Ctrl Pts',(20.7999688277064,-19.4152913566914,-15.3152771314083));
#81856=CARTESIAN_POINT('Ctrl Pts',(20.8181177584978,-19.3277377675104,-15.3101329516797));
#81857=CARTESIAN_POINT('Ctrl Pts',(20.827192324167,-19.2733599861546,-15.3070253234151));
#81858=CARTESIAN_POINT('Ctrl Pts',(20.8479099511833,-19.1102105665311,-15.2978807920945));
#81859=CARTESIAN_POINT('Ctrl Pts',(20.8532599347427,-19.0008270167028,-15.2919926180276));
#81860=CARTESIAN_POINT('Ctrl Pts',(20.8488264569386,-18.8457035655288,-15.2835435935355));
#81861=CARTESIAN_POINT('Ctrl Pts',(20.8460294166224,-18.799942842889,-15.2810373870488));
#81862=CARTESIAN_POINT('Ctrl Pts',(20.8396445421111,-18.7318678535178,-15.2772457724828));
#81863=CARTESIAN_POINT('Ctrl Pts',(20.8371813577142,-18.7094608772383,-15.2759874206289));
#81864=CARTESIAN_POINT('Ctrl Pts',(20.8335646191318,-18.6807843904216,-15.2743590646324));
#81865=CARTESIAN_POINT('Ctrl Pts',(20.832739865342,-18.6744743740556,-15.273999642275));
#81866=CARTESIAN_POINT('Ctrl Pts',(20.8258023941404,-18.6231974214837,-15.2710691176888));
#81867=CARTESIAN_POINT('Ctrl Pts',(20.8182741464527,-18.578437396997,-15.2684500502094));
#81868=CARTESIAN_POINT('Ctrl Pts',(20.8078120118602,-18.526499567822,-15.2653035776034));
#81869=CARTESIAN_POINT('Ctrl Pts',(20.8062695433121,-18.5190498709481,-15.2648496596602));
#81870=CARTESIAN_POINT('Ctrl Pts',(20.8037293599071,-18.5071061163287,-15.2641174950169));
#81871=CARTESIAN_POINT('Ctrl Pts',(20.8027570659559,-18.5026066398684,-15.2638406631855));
#81872=CARTESIAN_POINT('Ctrl Pts',(20.8010019881233,-18.4946110884284,-15.2633468806029));
#81873=CARTESIAN_POINT('Ctrl Pts',(20.8002249966559,-18.4911137902387,-15.2631302638108));
#81874=CARTESIAN_POINT('Ctrl Pts',(20.7985511656071,-18.4836690587019,-15.2626677798618));
#81875=CARTESIAN_POINT('Ctrl Pts',(20.7976518945992,-18.4797222816298,-15.2624217805373));
#81876=CARTESIAN_POINT('Ctrl Pts',(20.7951756506108,-18.4689965017218,-15.2617510760597));
#81877=CARTESIAN_POINT('Ctrl Pts',(20.7935765735611,-18.4622227276084,-15.2613251317179));
#81878=CARTESIAN_POINT('Ctrl Pts',(20.7852143222332,-18.4275650067871,-15.2591341058772));
#81879=CARTESIAN_POINT('Ctrl Pts',(20.7779185197208,-18.3998142035234,-15.2573408876463));
#81880=CARTESIAN_POINT('Ctrl Pts',(20.7547512141243,-18.3184553916971,-15.2519855954401));
#81881=CARTESIAN_POINT('Ctrl Pts',(20.737318225969,-18.2653199675577,-15.2483615798352));
#81882=CARTESIAN_POINT('Ctrl Pts',(20.6690492547427,-18.0820704260946,-15.2355500629643));
#81883=CARTESIAN_POINT('Ctrl Pts',(20.6074582691765,-17.956333248364,-15.2262198423816));
#81884=CARTESIAN_POINT('Ctrl Pts',(20.4869333088051,-17.7616704259775,-15.211445076017));
#81885=CARTESIAN_POINT('Ctrl Pts',(20.4351764773242,-17.6888048920255,-15.2058201901091));
#81886=CARTESIAN_POINT('Ctrl Pts',(20.3703433829837,-17.6087736734458,-15.1995360879001));
#81887=CARTESIAN_POINT('Ctrl Pts',(20.3616177711602,-17.5982138144338,-15.1987045115429));
#81888=CARTESIAN_POINT('Ctrl Pts',(20.3474530788473,-17.5814064241127,-15.1973768501526));
#81889=CARTESIAN_POINT('Ctrl Pts',(20.3420788674547,-17.5751049615185,-15.1968781383255));
#81890=CARTESIAN_POINT('Ctrl Pts',(20.3324668673792,-17.5639675744327,-15.1959949566643));
#81891=CARTESIAN_POINT('Ctrl Pts',(20.3282437901353,-17.5591191438014,-15.195609887017));
#81892=CARTESIAN_POINT('Ctrl Pts',(20.3193946534816,-17.549052595502,-15.1948091032061));
#81893=CARTESIAN_POINT('Ctrl Pts',(20.3147647625277,-17.5438379374466,-15.1943935553569));
#81894=CARTESIAN_POINT('Ctrl Pts',(20.302665057392,-17.5303448856863,-15.1933163496394));
#81895=CARTESIAN_POINT('Ctrl Pts',(20.29515539482,-17.5221023929127,-15.1926563761632));
#81896=CARTESIAN_POINT('Ctrl Pts',(20.2621732122885,-17.4864712255106,-15.1897943605675));
#81897=CARTESIAN_POINT('Ctrl Pts',(20.2360415735037,-17.4596999900685,-15.1876206357482));
#81898=CARTESIAN_POINT('Ctrl Pts',(20.1646403548181,-17.3903280428261,-15.181908265251));
#81899=CARTESIAN_POINT('Ctrl Pts',(20.1181803061272,-17.349003781144,-15.1784214398209));
#81900=CARTESIAN_POINT('Ctrl Pts',(19.9663676309826,-17.2255021967237,-15.167597607391));
#81901=CARTESIAN_POINT('Ctrl Pts',(19.855030535987,-17.1512185487875,-15.1604808644335));
#81902=CARTESIAN_POINT('Ctrl Pts',(19.6640639489695,-17.0484206722914,-15.1485261417979));
#81903=CARTESIAN_POINT('Ctrl Pts',(19.5884279754497,-17.0132935445388,-15.1438419294371));
#81904=CARTESIAN_POINT('Ctrl Pts',(19.5020093978761,-16.9791993224962,-15.1383369991295));
#81905=CARTESIAN_POINT('Ctrl Pts',(19.4930659005399,-16.9757409331756,-15.1377655029824));
#81906=CARTESIAN_POINT('Ctrl Pts',(19.4797988862489,-16.9707140108053,-15.1369146581061));
#81907=CARTESIAN_POINT('Ctrl Pts',(19.4754931123857,-16.9690985619355,-15.1366380421839));
#81908=CARTESIAN_POINT('Ctrl Pts',(19.4678322038706,-16.9662527685321,-15.1361449790827));
#81909=CARTESIAN_POINT('Ctrl Pts',(19.4644791830265,-16.9650168763513,-15.1359288669445));
#81910=CARTESIAN_POINT('Ctrl Pts',(19.4572740091007,-16.9623818195544,-15.1354637935784));
#81911=CARTESIAN_POINT('Ctrl Pts',(19.4534209749595,-16.9609853701365,-15.1352146811577));
#81912=CARTESIAN_POINT('Ctrl Pts',(19.4427991126033,-16.9571705627356,-15.1345268599629));
#81913=CARTESIAN_POINT('Ctrl Pts',(19.4360220584232,-16.9547755028851,-15.1340868053146));
#81914=CARTESIAN_POINT('Ctrl Pts',(19.3992330326576,-16.9419843751326,-15.1316919738592));
#81915=CARTESIAN_POINT('Ctrl Pts',(19.3690038942946,-16.9322308046017,-15.1297025917515));
#81916=CARTESIAN_POINT('Ctrl Pts',(19.1820076956383,-16.8765082501724,-15.1173129046644));
#81917=CARTESIAN_POINT('Ctrl Pts',(19.0205774493177,-16.8481344881915,-15.1063100349775));
#81918=CARTESIAN_POINT('Ctrl Pts',(18.7406727451833,-16.8317788387786,-15.0879942660418));
#81919=CARTESIAN_POINT('Ctrl Pts',(18.6234743744695,-16.8346492426108,-15.0805396456059));
#81920=CARTESIAN_POINT('Ctrl Pts',(18.4928870449473,-16.848726882749,-15.0725197636851));
#81921=CARTESIAN_POINT('Ctrl Pts',(18.4786929316005,-16.8504026124406,-15.0716516208191));
#81922=CARTESIAN_POINT('Ctrl Pts',(18.4561300844777,-16.8532983055921,-15.0702770988864));
#81923=CARTESIAN_POINT('Ctrl Pts',(18.4477500014746,-16.8544248681758,-15.0697677903367));
#81924=CARTESIAN_POINT('Ctrl Pts',(18.4329827849576,-16.8565002202061,-15.0688723564639));
#81925=CARTESIAN_POINT('Ctrl Pts',(18.4265928636803,-16.8574280759924,-15.0684855747564));
#81926=CARTESIAN_POINT('Ctrl Pts',(18.4133856892092,-16.859407578504,-15.0676875167435));
#81927=CARTESIAN_POINT('Ctrl Pts',(18.4065691230234,-16.8604633397141,-15.067276375684));
#81928=CARTESIAN_POINT('Ctrl Pts',(18.3890861295657,-16.8632587002088,-15.0662237703251));
#81929=CARTESIAN_POINT('Ctrl Pts',(18.3784275594396,-16.865046708347,-15.0655838467272));
#81930=CARTESIAN_POINT('Ctrl Pts',(18.3340075361081,-16.8728484899745,-15.0629240090824));
#81931=CARTESIAN_POINT('Ctrl Pts',(18.3003799080524,-16.8796007177522,-15.0609276050943));
#81932=CARTESIAN_POINT('Ctrl Pts',(18.2132099163893,-16.8993187867546,-15.0557858138884));
#81933=CARTESIAN_POINT('Ctrl Pts',(18.159982371913,-16.9135626373115,-15.0526797697658));
#81934=CARTESIAN_POINT('Ctrl Pts',(18.0045299079525,-16.9617352896282,-15.0436303373786));
#81935=CARTESIAN_POINT('Ctrl Pts',(17.9042699295139,-17.0014028728595,-15.0378294711641));
#81936=CARTESIAN_POINT('Ctrl Pts',(17.6993569682821,-17.1011465049066,-15.0254258979975));
#81937=CARTESIAN_POINT('Ctrl Pts',(17.5959457510176,-17.1628748053974,-15.0188285157138));
#81938=CARTESIAN_POINT('Ctrl Pts',(17.4906332544539,-17.2385769950746,-15.0111418617979));
#81939=CARTESIAN_POINT('Ctrl Pts',(17.4829566618978,-17.2441739502166,-15.0105755764535));
#81940=CARTESIAN_POINT('Ctrl Pts',(17.4716343678639,-17.2525462638494,-15.0097310289831));
#81941=CARTESIAN_POINT('Ctrl Pts',(17.4679594639195,-17.2552821829749,-15.0094554414432));
#81942=CARTESIAN_POINT('Ctrl Pts',(17.4615604238182,-17.2600785504742,-15.0089729369825));
#81943=CARTESIAN_POINT('Ctrl Pts',(17.4588323581629,-17.2621336882941,-15.0087663927705));
#81944=CARTESIAN_POINT('Ctrl Pts',(17.452943447302,-17.2665923708874,-15.0083187004817));
#81945=CARTESIAN_POINT('Ctrl Pts',(17.449784434805,-17.2689981732058,-15.0080773971103));
#81946=CARTESIAN_POINT('Ctrl Pts',(17.4413944857164,-17.275425063839,-15.0074335109115));
#81947=CARTESIAN_POINT('Ctrl Pts',(17.4361755967001,-17.2794617051716,-15.0070298542132));
#81948=CARTESIAN_POINT('Ctrl Pts',(17.4245780164326,-17.2885190220691,-15.0061259843416));
#81949=CARTESIAN_POINT('Ctrl Pts',(17.4182091937257,-17.2935520977632,-15.005624956281));
#81950=CARTESIAN_POINT('Ctrl Pts',(17.3989854179596,-17.3089244640379,-15.0040988344534));
#81951=CARTESIAN_POINT('Ctrl Pts',(17.386222530684,-17.3193772607058,-15.0030667305062));
#81952=CARTESIAN_POINT('Ctrl Pts',(17.3390421698338,-17.3589481986043,-14.9991842798635));
#81953=CARTESIAN_POINT('Ctrl Pts',(17.3054371382018,-17.389012789395,-14.9962835857847));
#81954=CARTESIAN_POINT('Ctrl Pts',(17.2178843621736,-17.4725250841375,-14.9884087002875));
#81955=CARTESIAN_POINT('Ctrl Pts',(17.1658090434186,-17.5278408855327,-14.9833808222618));
#81956=CARTESIAN_POINT('Ctrl Pts',(17.0169246971401,-17.704080583839,-14.9681409955478));
#81957=CARTESIAN_POINT('Ctrl Pts',(16.9302842240295,-17.8329484910158,-14.9580560622777));
#81958=CARTESIAN_POINT('Ctrl Pts',(16.8473597513694,-17.9913486797774,-14.9470407091089));
#81959=CARTESIAN_POINT('Ctrl Pts',(16.8366142124931,-18.0127504942487,-14.9455780235587));
#81960=CARTESIAN_POINT('Ctrl Pts',(16.8220268664709,-18.0430765031995,-14.9435403616427));
#81961=CARTESIAN_POINT('Ctrl Pts',(16.8178801298435,-18.0518512153695,-14.9429548176323));
#81962=CARTESIAN_POINT('Ctrl Pts',(16.8112693089261,-18.0660927587062,-14.9420109046922));
#81963=CARTESIAN_POINT('Ctrl Pts',(16.8087678885144,-18.0715420120025,-14.9416512481585));
#81964=CARTESIAN_POINT('Ctrl Pts',(16.8036027000191,-18.0829214504145,-14.9409033115526));
#81965=CARTESIAN_POINT('Ctrl Pts',(16.8009430254914,-18.0888534331407,-14.9405151754291));
#81966=CARTESIAN_POINT('Ctrl Pts',(16.7947203172894,-18.1029052254155,-14.9395998444167));
#81967=CARTESIAN_POINT('Ctrl Pts',(16.7911808725664,-18.1110353956771,-14.9390734615493));
#81968=CARTESIAN_POINT('Ctrl Pts',(16.7796053354061,-18.1380877733401,-14.9373324198111));
#81969=CARTESIAN_POINT('Ctrl Pts',(16.7717936293248,-18.1571051512969,-14.9361253861798));
#81970=CARTESIAN_POINT('Ctrl Pts',(16.7318168056899,-18.2586098969516,-14.929767399564));
#81971=CARTESIAN_POINT('Ctrl Pts',(16.7045710054868,-18.3429450653894,-14.9247836181472));
#81972=CARTESIAN_POINT('Ctrl Pts',(16.6389736200311,-18.6001072463063,-14.9101349325607));
#81973=CARTESIAN_POINT('Ctrl Pts',(16.6169140090866,-18.7762389717622,-14.9008598182712));
#81974=CARTESIAN_POINT('Ctrl Pts',(16.6170002518852,-18.9530327061848,-14.8907771671312));
#81975=CARTESIAN_POINT('Ctrl Pts',(16.6170002532685,-18.9530355380041,-14.8907770056308));
#81976=CARTESIAN_POINT('Ctrl Pts',(16.6170133611375,-18.9798325798375,-14.8892487531684));
#81977=CARTESIAN_POINT('Ctrl Pts',(16.6175352642842,-19.0066259871557,-14.8877018039767));
#81978=CARTESIAN_POINT('Ctrl Pts',(16.6191227654136,-19.0478815541535,-14.8852809856311));
#81979=CARTESIAN_POINT('Ctrl Pts',(16.6198286097373,-19.0623553210824,-14.8844242982576));
#81980=CARTESIAN_POINT('Ctrl Pts',(16.6209600190508,-19.0815110785819,-14.8832793646105));
#81981=CARTESIAN_POINT('Ctrl Pts',(16.6212526903976,-19.0862009142593,-14.8829981706578));
#81982=CARTESIAN_POINT('Ctrl Pts',(16.6217938179313,-19.0944311792435,-14.8825030866471));
#81983=CARTESIAN_POINT('Ctrl Pts',(16.6220355693814,-19.0979720513336,-14.8822895645769));
#81984=CARTESIAN_POINT('Ctrl Pts',(16.6225281743406,-19.1049296119789,-14.8818689494618));
#81985=CARTESIAN_POINT('Ctrl Pts',(16.6227784202662,-19.108346339654,-14.8816618899991));
#81986=CARTESIAN_POINT('Ctrl Pts',(16.6233330673721,-19.1156749674767,-14.8812166601339));
#81987=CARTESIAN_POINT('Ctrl Pts',(16.6236400494739,-19.1195866167188,-14.8809783487989));
#81988=CARTESIAN_POINT('Ctrl Pts',(16.6244765273345,-19.1298783411693,-14.8803496173194));
#81989=CARTESIAN_POINT('Ctrl Pts',(16.625024088128,-19.1362568497938,-14.8799582038806));
#81990=CARTESIAN_POINT('Ctrl Pts',(16.627416796096,-19.1627202247775,-14.8783273285818));
#81991=CARTESIAN_POINT('Ctrl Pts',(16.6295199328799,-19.1827799525984,-14.8770744345601));
#81992=CARTESIAN_POINT('Ctrl Pts',(16.6324142606028,-19.2070383307557,-14.8755415570272));
#81993=CARTESIAN_POINT('Ctrl Pts',(16.6329320449516,-19.2112693924791,-14.8752735421504));
#81994=CARTESIAN_POINT('Ctrl Pts',(16.6366907709949,-19.241232883062,-14.8733710028631));
#81995=CARTESIAN_POINT('Ctrl Pts',(16.6403914468671,-19.2669043921709,-14.8717174068611));
#81996=CARTESIAN_POINT('Ctrl Pts',(16.6659945805772,-19.4240148036282,-14.861477304345));
#81997=CARTESIAN_POINT('Ctrl Pts',(16.6997789103089,-19.5531158497064,-14.8525677425466));
#81998=CARTESIAN_POINT('Ctrl Pts',(16.7454194444943,-19.6781104421951,-14.843838520965));
#81999=CARTESIAN_POINT('Origin',(18.734,-18.952,0.));
#82000=CARTESIAN_POINT('',(16.7454194457665,-19.6781104456791,-14.0426552583743));
#82001=CARTESIAN_POINT('',(16.7454194499637,-19.6781104571739,-14.2664527091733));
#82002=CARTESIAN_POINT('',(16.7454194499637,-19.6781104571739,0.));
#82003=CARTESIAN_POINT('',(16.6195738444081,-18.9515327933745,-14.3109440134329));
#82004=CARTESIAN_POINT('Ctrl Pts',(16.7454194499637,-19.6781104571739,-14.2664527091733));
#82005=CARTESIAN_POINT('Ctrl Pts',(16.719650694312,-19.6075382105118,-14.2709758243854));
#82006=CARTESIAN_POINT('Ctrl Pts',(16.6976093484952,-19.5355011702686,-14.2754989395975));
#82007=CARTESIAN_POINT('Ctrl Pts',(16.6794520904527,-19.4624134474864,-14.2800220548096));
#82008=CARTESIAN_POINT('Ctrl Pts',(16.6613181208718,-19.3894194668659,-14.2845393686835));
#82009=CARTESIAN_POINT('Ctrl Pts',(16.6470584424874,-19.31537790376,-14.2890566825574));
#82010=CARTESIAN_POINT('Ctrl Pts',(16.6367803548254,-19.2407191713304,-14.2935739964313));
#82011=CARTESIAN_POINT('Ctrl Pts',(16.6265157658079,-19.1661584913522,-14.298085377527));
#82012=CARTESIAN_POINT('Ctrl Pts',(16.620222420087,-19.0909826864512,-14.3025967586227));
#82013=CARTESIAN_POINT('Ctrl Pts',(16.6179565327474,-19.0156321042995,-14.3071081397184));
#82014=CARTESIAN_POINT('Ctrl Pts',(16.6173143794296,-18.9942777211936,-14.3083866668048));
#82015=CARTESIAN_POINT('Ctrl Pts',(16.6169953775011,-18.9729093504981,-14.3096651938911));
#82016=CARTESIAN_POINT('Ctrl Pts',(16.617000050606,-18.9515371115436,-14.3109437209775));
#82017=CARTESIAN_POINT('Ctrl Pts',(16.6203928623232,-18.9515314192714,-14.3109441064964));
#82018=CARTESIAN_POINT('Ctrl Pts',(16.6197600125371,-18.626044201896,-14.3304466040356));
#82019=CARTESIAN_POINT('Ctrl Pts',(16.8436652651824,-17.5938832267072,-14.3923410371352));
#82020=CARTESIAN_POINT('Ctrl Pts',(18.4531255181642,-16.4645434415686,-14.4966274057954));
#82021=CARTESIAN_POINT('Ctrl Pts',(20.6735252872927,-17.3694159533938,-14.6238032124768));
#82022=CARTESIAN_POINT('Ctrl Pts',(21.1145309858464,-19.7262111017335,-14.7509790191583));
#82023=CARTESIAN_POINT('Ctrl Pts',(19.3715472573024,-21.3727156171948,-14.8781548258396));
#82024=CARTESIAN_POINT('Ctrl Pts',(17.4471161530942,-20.8979085117977,-14.9832889524932));
#82025=CARTESIAN_POINT('Ctrl Pts',(16.864829023637,-19.9961148353166,-15.0460311435864));
#82026=CARTESIAN_POINT('Ctrl Pts',(16.7486736625677,-19.6769293383554,-15.066381399119));
#82027=CARTESIAN_POINT('Ctrl Pts',(16.7454194444943,-19.6781104421951,-14.843838520965));
#82028=CARTESIAN_POINT('Ctrl Pts',(16.7603648243346,-19.7190409811572,-14.8409800633554));
#82029=CARTESIAN_POINT('Ctrl Pts',(16.7765815379704,-19.7595310236544,-14.8381385948187));
#82030=CARTESIAN_POINT('Ctrl Pts',(16.8176696080674,-19.8535803150628,-14.8315214728077));
#82031=CARTESIAN_POINT('Ctrl Pts',(16.8435379478377,-19.9066326300905,-14.8277759596819));
#82032=CARTESIAN_POINT('Ctrl Pts',(16.8887248800872,-19.9902424674523,-14.8218599513893));
#82033=CARTESIAN_POINT('Ctrl Pts',(16.9066665112555,-20.0215046801535,-14.8196445490687));
#82034=CARTESIAN_POINT('Ctrl Pts',(16.9311172384433,-20.0616953709696,-14.8167901621556));
#82035=CARTESIAN_POINT('Ctrl Pts',(16.9369093018647,-20.0710509810126,-14.8161252487326));
#82036=CARTESIAN_POINT('Ctrl Pts',(16.9464736002627,-20.0862339024914,-14.8150452937432));
#82037=CARTESIAN_POINT('Ctrl Pts',(16.9502019638814,-20.0920884805326,-14.8146286419104));
#82038=CARTESIAN_POINT('Ctrl Pts',(16.9574453386305,-20.1033400956848,-14.8138274356015));
#82039=CARTESIAN_POINT('Ctrl Pts',(16.9609563133272,-20.108739628149,-14.8134427369955));
#82040=CARTESIAN_POINT('Ctrl Pts',(16.9690774761028,-20.1211053261279,-14.8125611979127));
#82041=CARTESIAN_POINT('Ctrl Pts',(16.9737043828028,-20.1280604244974,-14.8120649903535));
#82042=CARTESIAN_POINT('Ctrl Pts',(16.9861632145533,-20.1465501035786,-14.8107446955642));
#82043=CARTESIAN_POINT('Ctrl Pts',(16.9940682038156,-20.1580351309188,-14.8099233705307));
#82044=CARTESIAN_POINT('Ctrl Pts',(17.0584921859535,-20.2496837138478,-14.8033574783419));
#82045=CARTESIAN_POINT('Ctrl Pts',(17.1204100857391,-20.3259143218483,-14.7978305945283));
#82046=CARTESIAN_POINT('Ctrl Pts',(17.2808130706187,-20.4975262899131,-14.7848753274666));
#82047=CARTESIAN_POINT('Ctrl Pts',(17.383690158982,-20.5881737878757,-14.7775972522211));
#82048=CARTESIAN_POINT('Ctrl Pts',(17.5362176301092,-20.6983227406158,-14.767172385556));
#82049=CARTESIAN_POINT('Ctrl Pts',(17.5789237557827,-20.7268588340156,-14.7642854493444));
#82050=CARTESIAN_POINT('Ctrl Pts',(17.6379503440067,-20.7632671002145,-14.7602785940892));
#82051=CARTESIAN_POINT('Ctrl Pts',(17.6533983727011,-20.7725255932984,-14.7592284419061));
#82052=CARTESIAN_POINT('Ctrl Pts',(17.6764325565737,-20.7859342467276,-14.7576575146448));
#82053=CARTESIAN_POINT('Ctrl Pts',(17.6839294305201,-20.7902370664145,-14.7571454454383));
#82054=CARTESIAN_POINT('Ctrl Pts',(17.6975505237689,-20.7979443594023,-14.7562132627727));
#82055=CARTESIAN_POINT('Ctrl Pts',(17.7036657369816,-20.8013645930733,-14.755794105828));
#82056=CARTESIAN_POINT('Ctrl Pts',(17.7133274982744,-20.8067056130249,-14.7551306521781));
#82057=CARTESIAN_POINT('Ctrl Pts',(17.7168628128953,-20.8086467646673,-14.7548876366302));
#82058=CARTESIAN_POINT('Ctrl Pts',(17.7204127123641,-20.8105827424277,-14.7546433437848));
#82059=CARTESIAN_POINT('Ctrl Pts',(17.720421805009,-20.8105877011177,-14.7546427180559));
#82060=CARTESIAN_POINT('Ctrl Pts',(17.7204400455879,-20.810597648476,-14.7546414627898));
#82061=CARTESIAN_POINT('Ctrl Pts',(17.7204491939729,-20.8106026373893,-14.7546408332214));
#82062=CARTESIAN_POINT('Ctrl Pts',(17.7204675464048,-20.8106126453942,-14.7546395702505));
#82063=CARTESIAN_POINT('Ctrl Pts',(17.7204767503375,-20.8106176644225,-14.7546389368558));
#82064=CARTESIAN_POINT('Ctrl Pts',(17.7204952147367,-20.8106277331299,-14.7546376661722));
#82065=CARTESIAN_POINT('Ctrl Pts',(17.72050447466,-20.8106327825117,-14.7546370289206));
#82066=CARTESIAN_POINT('Ctrl Pts',(17.7205230511052,-20.8106429119579,-14.7546357505187));
#82067=CARTESIAN_POINT('Ctrl Pts',(17.720532367803,-20.8106479921173,-14.7546351093562));
#82068=CARTESIAN_POINT('Ctrl Pts',(17.7205510577489,-20.8106581830891,-14.7546338231357));
#82069=CARTESIAN_POINT('Ctrl Pts',(17.7205604314918,-20.8106632941703,-14.7546331780436));
#82070=CARTESIAN_POINT('Ctrl Pts',(17.7205792364403,-20.8106735474799,-14.7546318839011));
#82071=CARTESIAN_POINT('Ctrl Pts',(17.7205886672233,-20.8106786894768,-14.7546312348797));
#82072=CARTESIAN_POINT('Ctrl Pts',(17.7206075862087,-20.8106890045909,-14.7546299328815));
#82073=CARTESIAN_POINT('Ctrl Pts',(17.7206170751273,-20.8106941780974,-14.7546292798553));
#82074=CARTESIAN_POINT('Ctrl Pts',(17.7206361112033,-20.8107045566741,-14.754627969791));
#82075=CARTESIAN_POINT('Ctrl Pts',(17.7206456578982,-20.8107097614909,-14.7546273127847));
#82076=CARTESIAN_POINT('Ctrl Pts',(17.7206648098499,-20.8107202028609,-14.7546259947378));
#82077=CARTESIAN_POINT('Ctrl Pts',(17.7206744153742,-20.8107254395587,-14.7546253336788));
#82078=CARTESIAN_POINT('Ctrl Pts',(17.7206936855275,-20.8107359449828,-14.7546240074892));
#82079=CARTESIAN_POINT('Ctrl Pts',(17.720703349874,-20.8107412135541,-14.754623342378));
#82080=CARTESIAN_POINT('Ctrl Pts',(17.7207227380599,-20.8107517829333,-14.754622008057));
#82081=CARTESIAN_POINT('Ctrl Pts',(17.720732461944,-20.8107570837644,-14.7546213388442));
#82082=CARTESIAN_POINT('Ctrl Pts',(17.7207519318875,-20.8107676973171,-14.7546199988883));
#82083=CARTESIAN_POINT('Ctrl Pts',(17.7207617345034,-20.8107730408685,-14.7546193242527));
#82084=CARTESIAN_POINT('Ctrl Pts',(17.7207813823703,-20.8107837510092,-14.7546179720433));
#82085=CARTESIAN_POINT('Ctrl Pts',(17.7207912257096,-20.8107891165563,-14.754617294601));
#82086=CARTESIAN_POINT('Ctrl Pts',(17.7208109749234,-20.8107998815346,-14.7546159354083));
#82087=CARTESIAN_POINT('Ctrl Pts',(17.7208208790707,-20.810805280023,-14.7546152537767));
#82088=CARTESIAN_POINT('Ctrl Pts',(17.7208407832878,-20.8108161290784,-14.7546138839076));
#82089=CARTESIAN_POINT('Ctrl Pts',(17.7208507320892,-20.8108215516989,-14.7546131991987));
#82090=CARTESIAN_POINT('Ctrl Pts',(17.7238600593233,-20.8124617623195,-14.7544060867814));
#82091=CARTESIAN_POINT('Ctrl Pts',(17.7268633259617,-20.814089253502,-14.7541991910801));
#82092=CARTESIAN_POINT('Ctrl Pts',(17.7339044377272,-20.8178828641191,-14.7537136688863));
#82093=CARTESIAN_POINT('Ctrl Pts',(17.7379453724887,-20.8200431403993,-14.7534346760457));
#82094=CARTESIAN_POINT('Ctrl Pts',(17.7503888885578,-20.8266435661868,-14.7525745597346));
#82095=CARTESIAN_POINT('Ctrl Pts',(17.7588142462784,-20.831040195631,-14.7519907948979));
#82096=CARTESIAN_POINT('Ctrl Pts',(17.8741011760019,-20.8902165104202,-14.7439870055941));
#82097=CARTESIAN_POINT('Ctrl Pts',(17.9853937251691,-20.9358576552603,-14.7360862314006));
#82098=CARTESIAN_POINT('Ctrl Pts',(18.2037608151379,-21.0044075249404,-14.7209657371144));
#82099=CARTESIAN_POINT('Ctrl Pts',(18.3099493811008,-21.0289484332123,-14.7137738165293));
#82100=CARTESIAN_POINT('Ctrl Pts',(18.4915205581074,-21.0563972714244,-14.7019767744359));
#82101=CARTESIAN_POINT('Ctrl Pts',(18.56602766924,-21.0636513867005,-14.6972711837737));
#82102=CARTESIAN_POINT('Ctrl Pts',(18.6595278891682,-21.0677730133359,-14.6915379531465));
#82103=CARTESIAN_POINT('Ctrl Pts',(18.6782963262363,-21.0683503196864,-14.6903955667553));
#82104=CARTESIAN_POINT('Ctrl Pts',(18.7056176640075,-21.0688269934401,-14.6887444451672));
#82105=CARTESIAN_POINT('Ctrl Pts',(18.7141658016438,-21.0689243456196,-14.6882295384946));
#82106=CARTESIAN_POINT('Ctrl Pts',(18.7291626118652,-21.0690042938966,-14.6873290803836));
#82107=CARTESIAN_POINT('Ctrl Pts',(18.7356110080278,-21.0690092080056,-14.6869428349968));
#82108=CARTESIAN_POINT('Ctrl Pts',(18.7481386224584,-21.0689615152518,-14.686194242766));
#82109=CARTESIAN_POINT('Ctrl Pts',(18.7542177832687,-21.068912185266,-14.6858317971254));
#82110=CARTESIAN_POINT('Ctrl Pts',(18.7687599338419,-21.0687315333882,-14.6849666927904));
#82111=CARTESIAN_POINT('Ctrl Pts',(18.7772225561527,-21.0685756426931,-14.6844648066311));
#82112=CARTESIAN_POINT('Ctrl Pts',(18.8078160897656,-21.0678285142056,-14.6826558412952));
#82113=CARTESIAN_POINT('Ctrl Pts',(18.8299388123231,-21.0669408775289,-14.6813580252488));
#82114=CARTESIAN_POINT('Ctrl Pts',(19.0370389701553,-21.0553749533222,-14.6692946754642));
#82115=CARTESIAN_POINT('Ctrl Pts',(19.2198718785134,-21.0208048170024,-14.6593824185648));
#82116=CARTESIAN_POINT('Ctrl Pts',(19.4721947441697,-20.9377522807815,-14.6449022032807));
#82117=CARTESIAN_POINT('Ctrl Pts',(19.5470101888736,-20.9083118402315,-14.6404846012247));
#82118=CARTESIAN_POINT('Ctrl Pts',(19.6527371167917,-20.859593545986,-14.6338261229747));
#82119=CARTESIAN_POINT('Ctrl Pts',(19.6851152236189,-20.8436581371412,-14.6317273597458));
#82120=CARTESIAN_POINT('Ctrl Pts',(19.7236833739933,-20.8234357088646,-14.6291357782312));
#82121=CARTESIAN_POINT('Ctrl Pts',(19.7302801466285,-20.8199321879646,-14.6286892129485));
#82122=CARTESIAN_POINT('Ctrl Pts',(19.740521771587,-20.8144232143,-14.6279905496319));
#82123=CARTESIAN_POINT('Ctrl Pts',(19.7441795619733,-20.8124417641328,-14.6277399511774));
#82124=CARTESIAN_POINT('Ctrl Pts',(19.7509617901697,-20.8087418863478,-14.627273257665));
#82125=CARTESIAN_POINT('Ctrl Pts',(19.7540877351511,-20.807026341369,-14.6270573464479));
#82126=CARTESIAN_POINT('Ctrl Pts',(19.7611571988505,-20.803123287429,-14.6265672199138));
#82127=CARTESIAN_POINT('Ctrl Pts',(19.7650980510639,-20.8009310816346,-14.6262927073956));
#82128=CARTESIAN_POINT('Ctrl Pts',(19.7752540268794,-20.7952389776896,-14.625581977329));
#82129=CARTESIAN_POINT('Ctrl Pts',(19.7814584620601,-20.7917202625182,-14.6251445942695));
#82130=CARTESIAN_POINT('Ctrl Pts',(19.8194275875443,-20.7699325368102,-14.6224488957712));
#82131=CARTESIAN_POINT('Ctrl Pts',(19.8507292590293,-20.7508738547591,-14.62014444956));
#82132=CARTESIAN_POINT('Ctrl Pts',(20.0248086127646,-20.63858735415,-14.6069247806826));
#82133=CARTESIAN_POINT('Ctrl Pts',(20.1564066682974,-20.5291893155738,-14.5954192527772));
#82134=CARTESIAN_POINT('Ctrl Pts',(20.3389522421585,-20.3358064534019,-14.5781370528099));
#82135=CARTESIAN_POINT('Ctrl Pts',(20.3996864295436,-20.2620705985389,-14.5720751384163));
#82136=CARTESIAN_POINT('Ctrl Pts',(20.4677006787844,-20.1670838172241,-14.5648989846308));
#82137=CARTESIAN_POINT('Ctrl Pts',(20.4798921257299,-20.1495005071177,-14.5635949026581));
#82138=CARTESIAN_POINT('Ctrl Pts',(20.4968364360452,-20.1242533366134,-14.561756024665));
#82139=CARTESIAN_POINT('Ctrl Pts',(20.5018098241219,-20.1167397198995,-14.561212917568));
#82140=CARTESIAN_POINT('Ctrl Pts',(20.5103026318101,-20.103729375589,-14.5602795359416));
#82141=CARTESIAN_POINT('Ctrl Pts',(20.5138448513444,-20.0982477485228,-14.5598884103319));
#82142=CARTESIAN_POINT('Ctrl Pts',(20.520575731305,-20.0877252012392,-14.5591416411905));
#82143=CARTESIAN_POINT('Ctrl Pts',(20.5237685422999,-20.0826870223598,-14.5587858456449));
#82144=CARTESIAN_POINT('Ctrl Pts',(20.5320093747557,-20.0695608193267,-14.5578633847655));
#82145=CARTESIAN_POINT('Ctrl Pts',(20.5370241641798,-20.0614520109078,-14.5572979507869));
#82146=CARTESIAN_POINT('Ctrl Pts',(20.5539060487257,-20.0337375688856,-14.5553801433624));
#82147=CARTESIAN_POINT('Ctrl Pts',(20.5655097617488,-20.0139728090187,-14.5540373891474));
#82148=CARTESIAN_POINT('Ctrl Pts',(20.6636497706736,-19.8404147437282,-14.5424506522843));
#82149=CARTESIAN_POINT('Ctrl Pts',(20.7309626796511,-19.6765520703348,-14.5329674239608));
#82150=CARTESIAN_POINT('Ctrl Pts',(20.7997627420294,-19.4229179205356,-14.5186659629901));
#82151=CARTESIAN_POINT('Ctrl Pts',(20.8172421375998,-19.3383149430912,-14.5139384772064));
#82152=CARTESIAN_POINT('Ctrl Pts',(20.8348591924054,-19.2156229324011,-14.5068603226297));
#82153=CARTESIAN_POINT('Ctrl Pts',(20.8392147258312,-19.1782232544804,-14.5046731474516));
#82154=CARTESIAN_POINT('Ctrl Pts',(20.8432447221691,-19.1331984581278,-14.5019835250189));
#82155=CARTESIAN_POINT('Ctrl Pts',(20.8438784760683,-19.1256634433039,-14.5015315143473));
#82156=CARTESIAN_POINT('Ctrl Pts',(20.8447998580103,-19.1139581199353,-14.5008261700625));
#82157=CARTESIAN_POINT('Ctrl Pts',(20.8451155321546,-19.1097899945857,-14.5005743827684));
#82158=CARTESIAN_POINT('Ctrl Pts',(20.8456774774977,-19.1020664283429,-14.500106620884));
#82159=CARTESIAN_POINT('Ctrl Pts',(20.8459271159594,-19.0985112902746,-14.4998908373885));
#82160=CARTESIAN_POINT('Ctrl Pts',(20.8464704976197,-19.0904828272899,-14.4994024745223));
#82161=CARTESIAN_POINT('Ctrl Pts',(20.8467590080591,-19.0860092152714,-14.4991296071245));
#82162=CARTESIAN_POINT('Ctrl Pts',(20.8475667945086,-19.0728322150687,-14.4983237595379));
#82163=CARTESIAN_POINT('Ctrl Pts',(20.8480465071021,-19.0641266197254,-14.4977886433611));
#82164=CARTESIAN_POINT('Ctrl Pts',(20.8510777413293,-19.0021506463171,-14.4939609374982));
#82165=CARTESIAN_POINT('Ctrl Pts',(20.851669007667,-18.9488080223078,-14.4905713326707));
#82166=CARTESIAN_POINT('Ctrl Pts',(20.8497712787356,-18.8777207368241,-14.4859754337134));
#82167=CARTESIAN_POINT('Ctrl Pts',(20.8490723514105,-18.8599432990661,-14.4848194812918));
#82168=CARTESIAN_POINT('Ctrl Pts',(20.845641339746,-18.7938944644273,-14.4805046307251));
#82169=CARTESIAN_POINT('Ctrl Pts',(20.8414800045263,-18.7457130557192,-14.4773173739823));
#82170=CARTESIAN_POINT('Ctrl Pts',(20.8225347878885,-18.5891286039126,-14.4668984051702));
#82171=CARTESIAN_POINT('Ctrl Pts',(20.8009993719172,-18.4817125638282,-14.4596657342549));
#82172=CARTESIAN_POINT('Ctrl Pts',(20.7562766412917,-18.3234125975831,-14.4490923551298));
#82173=CARTESIAN_POINT('Ctrl Pts',(20.7392311382289,-18.2709905730079,-14.4456032688615));
#82174=CARTESIAN_POINT('Ctrl Pts',(20.7082857825986,-18.1871069811851,-14.4400457704914));
#82175=CARTESIAN_POINT('Ctrl Pts',(20.6956323614549,-18.1552162298279,-14.4379389208695));
#82176=CARTESIAN_POINT('Ctrl Pts',(20.6779797093515,-18.1136989138682,-14.4352024097579));
#82177=CARTESIAN_POINT('Ctrl Pts',(20.6736743539742,-18.1037846802256,-14.4345494073186));
#82178=CARTESIAN_POINT('Ctrl Pts',(20.6664971874799,-18.087597777187,-14.4334839101279));
#82179=CARTESIAN_POINT('Ctrl Pts',(20.6636703499423,-18.0813054928809,-14.4330698859469));
#82180=CARTESIAN_POINT('Ctrl Pts',(20.6581380598985,-18.0691504001565,-14.4322703711206));
#82181=CARTESIAN_POINT('Ctrl Pts',(20.6554364441083,-18.0632859390265,-14.4318847541351));
#82182=CARTESIAN_POINT('Ctrl Pts',(20.6491353941242,-18.0497711469525,-14.4309963328076));
#82183=CARTESIAN_POINT('Ctrl Pts',(20.6455168604704,-18.0421298024447,-14.4304941945357));
#82184=CARTESIAN_POINT('Ctrl Pts',(20.6356595183159,-18.0216321826915,-14.4291475809847));
#82185=CARTESIAN_POINT('Ctrl Pts',(20.6293360886682,-18.0088169186273,-14.428306047138));
#82186=CARTESIAN_POINT('Ctrl Pts',(20.5701243777261,-17.8918171469568,-14.4206240394106));
#82187=CARTESIAN_POINT('Ctrl Pts',(20.5088228373494,-17.7921079481606,-14.4141002663022));
#82188=CARTESIAN_POINT('Ctrl Pts',(20.3431641823924,-17.5667992185879,-14.3987907175919));
#82189=CARTESIAN_POINT('Ctrl Pts',(20.2319364432361,-17.4472192493636,-14.3901881689856));
#82190=CARTESIAN_POINT('Ctrl Pts',(20.0834401150863,-17.3205118968985,-14.3789789594798));
#82191=CARTESIAN_POINT('Ctrl Pts',(20.0582748973489,-17.3000200391511,-14.37708619202));
#82192=CARTESIAN_POINT('Ctrl Pts',(20.0269359738743,-17.275677261837,-14.3747234396652));
#82193=CARTESIAN_POINT('Ctrl Pts',(20.0211990300786,-17.2712680140642,-14.3742906854574));
#82194=CARTESIAN_POINT('Ctrl Pts',(20.0121690986088,-17.264401221301,-14.3736089816574));
#82195=CARTESIAN_POINT('Ctrl Pts',(20.008891305515,-17.2619236582429,-14.3733614159221));
#82196=CARTESIAN_POINT('Ctrl Pts',(20.0027504788832,-17.2573100631652,-14.3728973571606));
#82197=CARTESIAN_POINT('Ctrl Pts',(19.9998892447891,-17.2551717296833,-14.3726810291808));
#82198=CARTESIAN_POINT('Ctrl Pts',(19.9933447615646,-17.2503064982866,-14.3721859905242));
#82199=CARTESIAN_POINT('Ctrl Pts',(19.9896580738096,-17.2475843221155,-14.3719069575251));
#82200=CARTESIAN_POINT('Ctrl Pts',(19.9782963268728,-17.2392519062185,-14.3710465970564));
#82201=CARTESIAN_POINT('Ctrl Pts',(19.9705924150494,-17.2336814692508,-14.3704626260879));
#82202=CARTESIAN_POINT('Ctrl Pts',(19.8655544284441,-17.158804264792,-14.3624954152205));
#82203=CARTESIAN_POINT('Ctrl Pts',(19.7625708943982,-17.0978150956803,-14.3546360500476));
#82204=CARTESIAN_POINT('Ctrl Pts',(19.556843475407,-16.9984126205601,-14.3395419538394));
#82205=CARTESIAN_POINT('Ctrl Pts',(19.4551535936839,-16.9586319949511,-14.3323351635132));
#82206=CARTESIAN_POINT('Ctrl Pts',(19.2789846315027,-16.9049719317662,-14.3205019713434));
#82207=CARTESIAN_POINT('Ctrl Pts',(19.2060032480531,-16.8869219753311,-14.3157754911845));
#82208=CARTESIAN_POINT('Ctrl Pts',(19.1137256608774,-16.869249032614,-14.3100197141104));
#82209=CARTESIAN_POINT('Ctrl Pts',(19.0951953656295,-16.8659556300437,-14.3088746530865));
#82210=CARTESIAN_POINT('Ctrl Pts',(19.0681794453542,-16.8615248597706,-14.3072204026436));
#82211=CARTESIAN_POINT('Ctrl Pts',(19.059727342264,-16.8601912335316,-14.3067050088074));
#82212=CARTESIAN_POINT('Ctrl Pts',(19.0448905868193,-16.8579423027054,-14.3058039888301));
#82213=CARTESIAN_POINT('Ctrl Pts',(19.0385094482317,-16.8570048701877,-14.3054176660695));
#82214=CARTESIAN_POINT('Ctrl Pts',(19.0261077014693,-16.8552408293307,-14.3046691344161));
#82215=CARTESIAN_POINT('Ctrl Pts',(19.0200876284462,-16.854410955626,-14.3043068257372));
#82216=CARTESIAN_POINT('Ctrl Pts',(19.0056833679515,-16.8524884772962,-14.3034423834016));
#82217=CARTESIAN_POINT('Ctrl Pts',(18.9972960028912,-16.8514201504345,-14.3029410195686));
#82218=CARTESIAN_POINT('Ctrl Pts',(18.9669815049474,-16.8477433113492,-14.3011359235911));
#82219=CARTESIAN_POINT('Ctrl Pts',(18.9450198075027,-16.8454275971789,-14.2998414020953));
#82220=CARTESIAN_POINT('Ctrl Pts',(18.7379169477376,-16.8268613869831,-14.2877476574487));
#82221=CARTESIAN_POINT('Ctrl Pts',(18.5514349710742,-16.8347127102277,-14.277807919148));
#82222=CARTESIAN_POINT('Ctrl Pts',(18.2607935942403,-16.8856768599577,-14.2617211681073));
#82223=CARTESIAN_POINT('Ctrl Pts',(18.1548602647907,-16.9128319320364,-14.2557001056844));
#82224=CARTESIAN_POINT('Ctrl Pts',(18.0403434106466,-16.9518328360542,-14.2485597694457));
#82225=CARTESIAN_POINT('Ctrl Pts',(18.0292094009874,-16.9557288899198,-14.2478586747539));
#82226=CARTESIAN_POINT('Ctrl Pts',(18.0134001814295,-16.9614096515108,-14.2468526015562));
#82227=CARTESIAN_POINT('Ctrl Pts',(18.0086976111573,-16.9631182846657,-14.2465519960793));
#82228=CARTESIAN_POINT('Ctrl Pts',(18.0005936490082,-16.9660953440076,-14.246031571634));
#82229=CARTESIAN_POINT('Ctrl Pts',(17.9971893464367,-16.9673558910936,-14.245812221688));
#82230=CARTESIAN_POINT('Ctrl Pts',(17.9905867573782,-16.9698200313216,-14.2453853497427));
#82231=CARTESIAN_POINT('Ctrl Pts',(17.9873881369865,-16.9710226141728,-14.2451778940369));
#82232=CARTESIAN_POINT('Ctrl Pts',(17.978748319879,-16.9742948172629,-14.2446157813056));
#82233=CARTESIAN_POINT('Ctrl Pts',(17.9733127727665,-16.9763791278095,-14.2442602575995));
#82234=CARTESIAN_POINT('Ctrl Pts',(17.9530676974896,-16.9842382231789,-14.2429292355584));
#82235=CARTESIAN_POINT('Ctrl Pts',(17.9383151876999,-16.9901571631857,-14.2419456158599));
#82236=CARTESIAN_POINT('Ctrl Pts',(17.8094123898518,-17.0435680510149,-14.2332389818716));
#82237=CARTESIAN_POINT('Ctrl Pts',(17.6995697006187,-17.1008049873945,-14.2250577701307));
#82238=CARTESIAN_POINT('Ctrl Pts',(17.4544602765674,-17.2571841821322,-14.2058446951504));
#82239=CARTESIAN_POINT('Ctrl Pts',(17.3246745757517,-17.3634644444438,-14.1949287562502));
#82240=CARTESIAN_POINT('Ctrl Pts',(17.1939622353427,-17.499269412077,-14.1833517496273));
#82241=CARTESIAN_POINT('Ctrl Pts',(17.1794267457231,-17.5148345513655,-14.182053821091));
#82242=CARTESIAN_POINT('Ctrl Pts',(17.1590898221214,-17.5372817192189,-14.1802220377878));
#82243=CARTESIAN_POINT('Ctrl Pts',(17.1530939476409,-17.5439851066563,-14.1796799588728));
#82244=CARTESIAN_POINT('Ctrl Pts',(17.1428229797148,-17.5556163691263,-14.17874778975));
#82245=CARTESIAN_POINT('Ctrl Pts',(17.1385276475629,-17.5605261308442,-14.1783568542898));
#82246=CARTESIAN_POINT('Ctrl Pts',(17.1303461923325,-17.5699655997979,-14.1776100709782));
#82247=CARTESIAN_POINT('Ctrl Pts',(17.1264564021841,-17.5744920325338,-14.1772540729282));
#82248=CARTESIAN_POINT('Ctrl Pts',(17.116390057836,-17.5863066448367,-14.1763302714904));
#82249=CARTESIAN_POINT('Ctrl Pts',(17.1102435591015,-17.5936203437504,-14.1757637067052));
#82250=CARTESIAN_POINT('Ctrl Pts',(17.0894464840566,-17.6187095861363,-14.1738378763305));
#82251=CARTESIAN_POINT('Ctrl Pts',(17.0750362860497,-17.6366829083594,-14.1724883413812));
#82252=CARTESIAN_POINT('Ctrl Pts',(16.9537663431868,-17.7931028226989,-14.1609878253909));
#82253=CARTESIAN_POINT('Ctrl Pts',(16.8641501657937,-17.9440600889061,-14.1515817989786));
#82254=CARTESIAN_POINT('Ctrl Pts',(16.7591127368294,-18.1844380736309,-14.1373097815625));
#82255=CARTESIAN_POINT('Ctrl Pts',(16.7291075131656,-18.2666280500326,-14.1325252744366));
#82256=CARTESIAN_POINT('Ctrl Pts',(16.6934927520533,-18.3867941073107,-14.1253702344575));
#82257=CARTESIAN_POINT('Ctrl Pts',(16.6836950221498,-18.4234390994714,-14.1231672792692));
#82258=CARTESIAN_POINT('Ctrl Pts',(16.6731275271715,-18.467695269505,-14.1204601664176));
#82259=CARTESIAN_POINT('Ctrl Pts',(16.6714072199851,-18.4750750151874,-14.1200072118277));
#82260=CARTESIAN_POINT('Ctrl Pts',(16.6687987127553,-18.4865430789206,-14.1193007098061));
#82261=CARTESIAN_POINT('Ctrl Pts',(16.6678829298504,-18.4906251481073,-14.1190487168597));
#82262=CARTESIAN_POINT('Ctrl Pts',(16.6662094767803,-18.498189409679,-14.1185807682855));
#82263=CARTESIAN_POINT('Ctrl Pts',(16.6654484970054,-18.5016708107583,-14.1183650050015));
#82264=CARTESIAN_POINT('Ctrl Pts',(16.6637510235548,-18.5095316599399,-14.1178769386893));
#82265=CARTESIAN_POINT('Ctrl Pts',(16.6628196397407,-18.5139121425429,-14.117604349186));
#82266=CARTESIAN_POINT('Ctrl Pts',(16.6601202353279,-18.5268090113293,-14.1168000651794));
#82267=CARTESIAN_POINT('Ctrl Pts',(16.6583908185769,-18.5353332564236,-14.1162662468071));
#82268=CARTESIAN_POINT('Ctrl Pts',(16.6465063460822,-18.5958221003902,-14.1124636611002));
#82269=CARTESIAN_POINT('Ctrl Pts',(16.6382522868145,-18.6481366127104,-14.1090992535617));
#82270=CARTESIAN_POINT('Ctrl Pts',(16.6301911556275,-18.7155650934305,-14.1047115443988));
#82271=CARTESIAN_POINT('Ctrl Pts',(16.6285718192705,-18.730448021496,-14.1037398707023));
#82272=CARTESIAN_POINT('Ctrl Pts',(16.6204362476909,-18.8133924644856,-14.0983107777663));
#82273=CARTESIAN_POINT('Ctrl Pts',(16.6170625895878,-18.8817198861515,-14.0937881860309));
#82274=CARTESIAN_POINT('Ctrl Pts',(16.616855711663,-19.1108585919565,-14.0786472531482));
#82275=CARTESIAN_POINT('Ctrl Pts',(16.6350247738316,-19.2711508353488,-14.0681492526916));
#82276=CARTESIAN_POINT('Ctrl Pts',(16.6765204048595,-19.4510311559526,-14.056777750078));
#82277=CARTESIAN_POINT('Ctrl Pts',(16.6822553156789,-19.4741093771815,-14.0553254705806));
#82278=CARTESIAN_POINT('Ctrl Pts',(16.6908695980634,-19.5064373734598,-14.0532997717922));
#82279=CARTESIAN_POINT('Ctrl Pts',(16.6934253017039,-19.5157708275043,-14.0527159490391));
#82280=CARTESIAN_POINT('Ctrl Pts',(16.6976666649319,-19.5308535538158,-14.0517740673681));
#82281=CARTESIAN_POINT('Ctrl Pts',(16.6993128687413,-19.536613690664,-14.0514147315572));
#82282=CARTESIAN_POINT('Ctrl Pts',(16.7027975173043,-19.5486135996585,-14.0506668844873));
#82283=CARTESIAN_POINT('Ctrl Pts',(16.7046403176142,-19.5548520498185,-14.0502785197106));
#82284=CARTESIAN_POINT('Ctrl Pts',(16.7090695303949,-19.5695958395848,-14.0493616204611));
#82285=CARTESIAN_POINT('Ctrl Pts',(16.7116808336213,-19.5780936198187,-14.0488339058202));
#82286=CARTESIAN_POINT('Ctrl Pts',(16.7205471772908,-19.6063124363643,-14.0470838241541));
#82287=CARTESIAN_POINT('Ctrl Pts',(16.7270378946957,-19.6259585938869,-14.0458691933702));
#82288=CARTESIAN_POINT('Ctrl Pts',(16.7375951449116,-19.6564073802206,-14.0439912496844));
#82289=CARTESIAN_POINT('Ctrl Pts',(16.741463193259,-19.667275555683,-14.0433218615717));
#82290=CARTESIAN_POINT('Ctrl Pts',(16.7454194457665,-19.6781104456791,-14.0426552583743));
#82291=CARTESIAN_POINT('Origin',(18.734,-18.952,0.));
#82292=CARTESIAN_POINT('',(16.7454194499637,-19.6781104571739,-13.2445592876386));
#82293=CARTESIAN_POINT('',(16.7454194853472,-19.6781105540779,-13.4647888353055));
#82294=CARTESIAN_POINT('',(16.7454194499637,-19.6781104571739,0.));
#82295=CARTESIAN_POINT('',(16.6170008950802,-18.9539467328105,-13.5109437209775));
#82296=CARTESIAN_POINT('Ctrl Pts',(16.7454194853472,-19.6781105540779,-13.4647888353055));
#82297=CARTESIAN_POINT('Ctrl Pts',(16.7297666895009,-19.6352426400322,-13.4673502476732));
#82298=CARTESIAN_POINT('Ctrl Pts',(16.7154972636532,-19.5918609431498,-13.4699562924166));
#82299=CARTESIAN_POINT('Ctrl Pts',(16.6982006735783,-19.5329117146061,-13.4735579116563));
#82300=CARTESIAN_POINT('Ctrl Pts',(16.6939331613312,-19.5177425018985,-13.4744900067255));
#82301=CARTESIAN_POINT('Ctrl Pts',(16.6883270791775,-19.4969265527102,-13.4757780818251));
#82302=CARTESIAN_POINT('Ctrl Pts',(16.6868416780363,-19.4913194321066,-13.476125935793));
#82303=CARTESIAN_POINT('Ctrl Pts',(16.6845188929854,-19.4824034704128,-13.4766805778664));
#82304=CARTESIAN_POINT('Ctrl Pts',(16.6836664223934,-19.4790985387891,-13.4768865000793));
#82305=CARTESIAN_POINT('Ctrl Pts',(16.6819231278139,-19.4722717633015,-13.4773125674383));
#82306=CARTESIAN_POINT('Ctrl Pts',(16.6810333782576,-19.4687496940318,-13.4775327754571));
#82307=CARTESIAN_POINT('Ctrl Pts',(16.678936164473,-19.4603569743768,-13.4780584152838));
#82308=CARTESIAN_POINT('Ctrl Pts',(16.6777369482887,-19.4554843021042,-13.478364318273));
#82309=CARTESIAN_POINT('Ctrl Pts',(16.6752325957493,-19.4451503867218,-13.4790145418689));
#82310=CARTESIAN_POINT('Ctrl Pts',(16.6739318427581,-19.4396881325614,-13.4793591005458));
#82311=CARTESIAN_POINT('Ctrl Pts',(16.6704195235729,-19.4246740382725,-13.4803084432271));
#82312=CARTESIAN_POINT('Ctrl Pts',(16.668252589932,-19.4151120370729,-13.4809155501542));
#82313=CARTESIAN_POINT('Ctrl Pts',(16.6336164616417,-19.2571922345215,-13.4909794322946));
#82314=CARTESIAN_POINT('Ctrl Pts',(16.6171414694287,-19.1057964096688,-13.5011355937932));
#82315=CARTESIAN_POINT('Ctrl Pts',(16.6170009071419,-18.953959805644,-13.5111420756604));
#82316=CARTESIAN_POINT('Ctrl Pts',(16.6170008950802,-18.9539467328105,-13.5109437209775));
#82317=CARTESIAN_POINT('Ctrl Pts',(16.6169347298129,-18.8819944798437,-13.5152699622426));
#82318=CARTESIAN_POINT('Ctrl Pts',(16.6205410702701,-18.8099473001284,-13.5195962035077));
#82319=CARTESIAN_POINT('Ctrl Pts',(16.6278222442379,-18.738214450598,-13.5239224447729));
#82320=CARTESIAN_POINT('Ctrl Pts',(16.6350987839402,-18.6665272570402,-13.5282459325052));
#82321=CARTESIAN_POINT('Ctrl Pts',(16.6460454699348,-18.5951544878199,-13.5325694202375));
#82322=CARTESIAN_POINT('Ctrl Pts',(16.6606126061973,-18.524502964665,-13.5368929079699));
#82323=CARTESIAN_POINT('Ctrl Pts',(16.675175543473,-18.4538718068595,-13.541215149454));
#82324=CARTESIAN_POINT('Ctrl Pts',(16.6933567603003,-18.3839619667448,-13.545537390938));
#82325=CARTESIAN_POINT('Ctrl Pts',(16.7150553040208,-18.3151708906014,-13.5498596324221));
#82326=CARTESIAN_POINT('Ctrl Pts',(16.7367551488127,-18.2463756896604,-13.5541821330731));
#82327=CARTESIAN_POINT('Ctrl Pts',(16.7619725873321,-18.1786998565911,-13.5585046337241));
#82328=CARTESIAN_POINT('Ctrl Pts',(16.7905571249902,-18.1125246926958,-13.5628271343751));
#82329=CARTESIAN_POINT('Ctrl Pts',(16.8191715095123,-18.0462804312642,-13.5671541484134));
#82330=CARTESIAN_POINT('Ctrl Pts',(16.8511598101655,-17.9815404195957,-13.5714811624517));
#82331=CARTESIAN_POINT('Ctrl Pts',(16.8863242283789,-17.9186640222249,-13.57580817649));
#82332=CARTESIAN_POINT('Ctrl Pts',(16.9215100988963,-17.8557492666598,-13.5801378302541));
#82333=CARTESIAN_POINT('Ctrl Pts',(16.9598756760654,-17.7947008039885,-13.5844674840182));
#82334=CARTESIAN_POINT('Ctrl Pts',(17.0011797410101,-17.7358491252997,-13.5887971377822));
#82335=CARTESIAN_POINT('Ctrl Pts',(17.04255259404,-17.6768994346044,-13.5931340021826));
#82336=CARTESIAN_POINT('Ctrl Pts',(17.0868733907411,-17.6201542127689,-13.597470866583));
#82337=CARTESIAN_POINT('Ctrl Pts',(17.1338612235983,-17.5659102134942,-13.6018077309834));
#82338=CARTESIAN_POINT('Ctrl Pts',(17.1504345250056,-17.5467775552112,-13.6033374069974));
#82339=CARTESIAN_POINT('Ctrl Pts',(17.1673393021153,-17.5279557221355,-13.6048670830114));
#82340=CARTESIAN_POINT('Ctrl Pts',(17.1845622179522,-17.5094565657968,-13.6063967590254));
#82341=CARTESIAN_POINT('Ctrl Pts',(17.2339699045479,-17.4563877052552,-13.6107849679563));
#82342=CARTESIAN_POINT('Ctrl Pts',(17.2862036327226,-17.405756540934,-13.6151731768872));
#82343=CARTESIAN_POINT('Ctrl Pts',(17.3409933109754,-17.3578791249304,-13.6195613858181));
#82344=CARTESIAN_POINT('Ctrl Pts',(17.3957016722616,-17.3100727669502,-13.6239430819193));
#82345=CARTESIAN_POINT('Ctrl Pts',(17.4529580928702,-17.2650123587825,-13.6283247780206));
#82346=CARTESIAN_POINT('Ctrl Pts',(17.5124544762696,-17.2229784462147,-13.6327064741219));
#82347=CARTESIAN_POINT('Ctrl Pts',(17.5718809466836,-17.1809939268393,-13.6370830213816));
#82348=CARTESIAN_POINT('Ctrl Pts',(17.6335417591182,-17.1420291152643,-13.6414595686412));
#82349=CARTESIAN_POINT('Ctrl Pts',(17.6970957742222,-17.106324344159,-13.6458361159008));
#82350=CARTESIAN_POINT('Ctrl Pts',(17.7606094842934,-17.0706422165006,-13.6502098876178));
#82351=CARTESIAN_POINT('Ctrl Pts',(17.826013595286,-17.0382162628695,-13.6545836593348));
#82352=CARTESIAN_POINT('Ctrl Pts',(17.8929392167485,-17.009242743193,-13.6589574310518));
#82353=CARTESIAN_POINT('Ctrl Pts',(17.9598444725197,-16.9802780402557,-13.6633298718153));
#82354=CARTESIAN_POINT('Ctrl Pts',(18.0282698771528,-16.9547638770617,-13.6677023125789));
#82355=CARTESIAN_POINT('Ctrl Pts',(18.0978247669418,-16.9328491703582,-13.6720747533424));
#82356=CARTESIAN_POINT('Ctrl Pts',(18.167381435257,-16.9109339032931,-13.6764473059098));
#82357=CARTESIAN_POINT('Ctrl Pts',(18.2380671853859,-16.8926184185034,-13.6808198584771));
#82358=CARTESIAN_POINT('Ctrl Pts',(18.3094759435911,-16.8780018501623,-13.6851924110445));
#82359=CARTESIAN_POINT('Ctrl Pts',(18.3809588124991,-16.8633701121953,-13.6895695016118));
#82360=CARTESIAN_POINT('Ctrl Pts',(18.4531657140474,-16.8524450521881,-13.6939465921791));
#82361=CARTESIAN_POINT('Ctrl Pts',(18.5256809453902,-16.8452745381786,-13.6983236827465));
#82362=CARTESIAN_POINT('Ctrl Pts',(18.5982357799922,-16.8381001080853,-13.7027031638054));
#82363=CARTESIAN_POINT('Ctrl Pts',(18.6710987974697,-16.8346843291133,-13.7070826448644));
#82364=CARTESIAN_POINT('Ctrl Pts',(18.7438524696376,-16.8350229267085,-13.7114621259233));
#82365=CARTESIAN_POINT('Ctrl Pts',(18.8167350972012,-16.8353621244656,-13.715849369583));
#82366=CARTESIAN_POINT('Ctrl Pts',(18.8895075103812,-16.8394689605671,-13.7202366132428));
#82367=CARTESIAN_POINT('Ctrl Pts',(18.9617560691,-16.8472871518927,-13.7246238569025));
#82368=CARTESIAN_POINT('Ctrl Pts',(19.0108781271733,-16.8526027686348,-13.7276067598372));
#82369=CARTESIAN_POINT('Ctrl Pts',(19.0597581560649,-16.8596329436867,-13.730589662772));
#82370=CARTESIAN_POINT('Ctrl Pts',(19.1082694567066,-16.8683466282089,-13.7335725657068));
#82371=CARTESIAN_POINT('Ctrl Pts',(19.1796354137562,-16.8811655060193,-13.7379607746377));
#82372=CARTESIAN_POINT('Ctrl Pts',(19.2504813367648,-16.8976801162964,-13.7423489835686));
#82373=CARTESIAN_POINT('Ctrl Pts',(19.3203952805283,-16.9178344278368,-13.7467371924995));
#82374=CARTESIAN_POINT('Ctrl Pts',(19.3902054604072,-16.9379588270371,-13.7511188886007));
#82375=CARTESIAN_POINT('Ctrl Pts',(19.4590859472333,-16.9617120714409,-13.755500584702));
#82376=CARTESIAN_POINT('Ctrl Pts',(19.5266340795877,-16.9889869547361,-13.7598822808032));
#82377=CARTESIAN_POINT('Ctrl Pts',(19.594102837511,-17.0162297878729,-13.7642588280629));
#82378=CARTESIAN_POINT('Ctrl Pts',(19.6602419060114,-17.0469858596158,-13.7686353753225));
#82379=CARTESIAN_POINT('Ctrl Pts',(19.7246645510869,-17.0810984132724,-13.7730119225822));
#82380=CARTESIAN_POINT('Ctrl Pts',(19.7890463402572,-17.1151893332433,-13.7773856942991));
#82381=CARTESIAN_POINT('Ctrl Pts',(19.8517134405357,-17.1526322864694,-13.7817594660161));
#82382=CARTESIAN_POINT('Ctrl Pts',(19.9123011549776,-17.1932233262354,-13.7861332377331));
#82383=CARTESIAN_POINT('Ctrl Pts',(19.9728704323746,-17.2338020140118,-13.7905056784966));
#82384=CARTESIAN_POINT('Ctrl Pts',(20.0313611796543,-17.2775266181305,-13.7948781192602));
#82385=CARTESIAN_POINT('Ctrl Pts',(20.0874367225444,-17.3241492580497,-13.7992505600237));
#82386=CARTESIAN_POINT('Ctrl Pts',(20.1435136992923,-17.3707730901148,-13.8036231125911));
#82387=CARTESIAN_POINT('Ctrl Pts',(20.1971749793956,-17.4202947951746,-13.8079956651584));
#82388=CARTESIAN_POINT('Ctrl Pts',(20.2481174066906,-17.4724265889262,-13.8123682177258));
#82389=CARTESIAN_POINT('Ctrl Pts',(20.2991127039582,-17.5246124870198,-13.8167453082931));
#82390=CARTESIAN_POINT('Ctrl Pts',(20.3473831767919,-17.5794135364602,-13.8211223988604));
#82391=CARTESIAN_POINT('Ctrl Pts',(20.3926635636812,-17.6365061070015,-13.8254994894278));
#82392=CARTESIAN_POINT('Ctrl Pts',(20.4379686798704,-17.6936298579146,-13.8298789704867));
#82393=CARTESIAN_POINT('Ctrl Pts',(20.4802801788313,-17.7530472284184,-13.8342584515457));
#82394=CARTESIAN_POINT('Ctrl Pts',(20.5193756547,-17.8144048296496,-13.8386379326046));
#82395=CARTESIAN_POINT('Ctrl Pts',(20.5585404270373,-17.8758711868171,-13.8430251762643));
#82396=CARTESIAN_POINT('Ctrl Pts',(20.5944775548132,-17.9392842223068,-13.8474124199241));
#82397=CARTESIAN_POINT('Ctrl Pts',(20.6270104676962,-18.0042656652878,-13.8517996635838));
#82398=CARTESIAN_POINT('Ctrl Pts',(20.6491297135926,-18.0484467849177,-13.8547825665186));
#82399=CARTESIAN_POINT('Ctrl Pts',(20.6696762814795,-18.0933524542016,-13.8577654694534));
#82400=CARTESIAN_POINT('Ctrl Pts',(20.6886076987149,-18.1388593331259,-13.8607483723882));
#82401=CARTESIAN_POINT('Ctrl Pts',(20.7164580900962,-18.2058054245265,-13.8651365813191));
#82402=CARTESIAN_POINT('Ctrl Pts',(20.7409194707722,-18.2743146794849,-13.86952479025));
#82403=CARTESIAN_POINT('Ctrl Pts',(20.7618159759921,-18.3440103886486,-13.8739129991809));
#82404=CARTESIAN_POINT('Ctrl Pts',(20.7826814673336,-18.4136026578242,-13.8782946952822));
#82405=CARTESIAN_POINT('Ctrl Pts',(20.7999924489197,-18.4843774273517,-13.8826763913835));
#82406=CARTESIAN_POINT('Ctrl Pts',(20.8136211113041,-18.555938093957,-13.8870580874847));
#82407=CARTESIAN_POINT('Ctrl Pts',(20.8272337589255,-18.6274146710837,-13.8914346347444));
#82408=CARTESIAN_POINT('Ctrl Pts',(20.8371725931962,-18.6996748392574,-13.895811182004));
#82409=CARTESIAN_POINT('Ctrl Pts',(20.8433600899069,-18.7723085669599,-13.9001877292637));
#82410=CARTESIAN_POINT('Ctrl Pts',(20.8495436625971,-18.8448962314078,-13.9045615009806));
#82411=CARTESIAN_POINT('Ctrl Pts',(20.8519805772149,-18.9178565058778,-13.9089352726976));
#82412=CARTESIAN_POINT('Ctrl Pts',(20.8506449171335,-18.9907723454651,-13.9133090444146));
#82413=CARTESIAN_POINT('Ctrl Pts',(20.8493096634979,-19.0636659965176,-13.9176814851781));
#82414=CARTESIAN_POINT('Ctrl Pts',(20.8442041231404,-19.1365147575252,-13.9220539259417));
#82415=CARTESIAN_POINT('Ctrl Pts',(20.8353544889708,-19.2089013656685,-13.9264263667052));
#82416=CARTESIAN_POINT('Ctrl Pts',(20.826504628515,-19.2812898247453,-13.9307989192726));
#82417=CARTESIAN_POINT('Ctrl Pts',(20.8139105446928,-19.3532156289256,-13.9351714718399));
#82418=CARTESIAN_POINT('Ctrl Pts',(20.7976501258782,-19.4242680996667,-13.9395440244072));
#82419=CARTESIAN_POINT('Ctrl Pts',(20.7813728313876,-19.4953943113422,-13.9439211149746));
#82420=CARTESIAN_POINT('Ctrl Pts',(20.7614217126853,-19.5656449087054,-13.9482982055419));
#82421=CARTESIAN_POINT('Ctrl Pts',(20.737925310568,-19.6346216738904,-13.9526752961092));
#82422=CARTESIAN_POINT('Ctrl Pts',(20.7144160761934,-19.703636109847,-13.9570547771682));
#82423=CARTESIAN_POINT('Ctrl Pts',(20.687357882489,-19.7713748802473,-13.9614342582271));
#82424=CARTESIAN_POINT('Ctrl Pts',(20.6569274894879,-19.8374596942672,-13.965813739286));
#82425=CARTESIAN_POINT('Ctrl Pts',(20.6264431588195,-19.9036616431763,-13.9702009829458));
#82426=CARTESIAN_POINT('Ctrl Pts',(20.5925749169667,-19.9682033538493,-13.9745882266055));
#82427=CARTESIAN_POINT('Ctrl Pts',(20.5555452556642,-20.0307316077539,-13.9789754702652));
#82428=CARTESIAN_POINT('Ctrl Pts',(20.530368654148,-20.0732447952009,-13.9819583732));
#82429=CARTESIAN_POINT('Ctrl Pts',(20.503731560257,-20.1148277943093,-13.9849412761349));
#82430=CARTESIAN_POINT('Ctrl Pts',(20.475714693788,-20.1553781306983,-13.9879241790697));
#82431=CARTESIAN_POINT('Ctrl Pts',(20.434498513999,-20.2150325519721,-13.9923123880006));
#82432=CARTESIAN_POINT('Ctrl Pts',(20.3901335538169,-20.2726834623513,-13.9967005969315));
#82433=CARTESIAN_POINT('Ctrl Pts',(20.3428413739374,-20.3279790817841,-14.0010888058624));
#82434=CARTESIAN_POINT('Ctrl Pts',(20.2956193834941,-20.3831926333494,-14.0054705019636));
#82435=CARTESIAN_POINT('Ctrl Pts',(20.2454791086756,-20.4360574697364,-14.0098521980649));
#82436=CARTESIAN_POINT('Ctrl Pts',(20.1926848492426,-20.4862514495969,-14.0142338941661));
#82437=CARTESIAN_POINT('Ctrl Pts',(20.1399526272657,-20.5363864475366,-14.0186104414258));
#82438=CARTESIAN_POINT('Ctrl Pts',(20.084572963737,-20.5838564928137,-14.0229869886854));
#82439=CARTESIAN_POINT('Ctrl Pts',(20.0268486678902,-20.6283744575526,-14.027363535945));
#82440=CARTESIAN_POINT('Ctrl Pts',(19.9691609799528,-20.6728641896452,-14.031737307662));
#82441=CARTESIAN_POINT('Ctrl Pts',(19.9091319910002,-20.7144052619584,-14.036111079379));
#82442=CARTESIAN_POINT('Ctrl Pts',(19.8470983416197,-20.7527501442131,-14.040484851096));
#82443=CARTESIAN_POINT('Ctrl Pts',(19.785083569287,-20.7910833579914,-14.0448572918595));
#82444=CARTESIAN_POINT('Ctrl Pts',(19.7210657576847,-20.8262220591674,-14.0492297326231));
#82445=CARTESIAN_POINT('Ctrl Pts',(19.6554099365357,-20.8579624153832,-14.0536021733866));
#82446=CARTESIAN_POINT('Ctrl Pts',(19.5897524365603,-20.8897035832033,-14.057974725954));
#82447=CARTESIAN_POINT('Ctrl Pts',(19.5224572790424,-20.9180460253879,-14.0623472785213));
#82448=CARTESIAN_POINT('Ctrl Pts',(19.4539119391452,-20.9428329412274,-14.0667198310886));
#82449=CARTESIAN_POINT('Ctrl Pts',(19.3852954603087,-20.9676455818632,-14.071096921656));
#82450=CARTESIAN_POINT('Ctrl Pts',(19.3154266631736,-20.9888951643123,-14.0754740122233));
#82451=CARTESIAN_POINT('Ctrl Pts',(19.2447099626412,-21.0064742232647,-14.0798511027906));
#82452=CARTESIAN_POINT('Ctrl Pts',(19.1739546410939,-21.0240628827937,-14.0842305838495));
#82453=CARTESIAN_POINT('Ctrl Pts',(19.102350968027,-21.0379769355906,-14.0886100649085));
#82454=CARTESIAN_POINT('Ctrl Pts',(19.0303127030113,-21.0481602472221,-14.0929895459674));
#82455=CARTESIAN_POINT('Ctrl Pts',(18.9581467506545,-21.0583616087051,-14.0973767896272));
#82456=CARTESIAN_POINT('Ctrl Pts',(18.8855451489727,-21.0648189809294,-14.1017640332869));
#82457=CARTESIAN_POINT('Ctrl Pts',(18.8129253294097,-21.0675282537413,-14.1061512769466));
#82458=CARTESIAN_POINT('Ctrl Pts',(18.7635508497359,-21.0693702981885,-14.1091341798814));
#82459=CARTESIAN_POINT('Ctrl Pts',(18.7141679744272,-21.069480806371,-14.1121170828162));
#82460=CARTESIAN_POINT('Ctrl Pts',(18.6649065603162,-21.0678721834252,-14.1150999857511));
#82461=CARTESIAN_POINT('Ctrl Pts',(18.5924370961486,-21.0655057056244,-14.119488194682));
#82462=CARTESIAN_POINT('Ctrl Pts',(18.5199478924753,-21.0594071393707,-14.1238764036129));
#82463=CARTESIAN_POINT('Ctrl Pts',(18.4478546672521,-21.0495723702763,-14.1282646125438));
#82464=CARTESIAN_POINT('Ctrl Pts',(18.3758684403282,-21.0397521976099,-14.132646308645));
#82465=CARTESIAN_POINT('Ctrl Pts',(18.3042774991944,-21.0262068946334,-14.1370280047463));
#82466=CARTESIAN_POINT('Ctrl Pts',(18.2334957741921,-21.0089843266171,-14.1414097008476));
#82467=CARTESIAN_POINT('Ctrl Pts',(18.1627972233499,-20.9917819964889,-14.1457862481072));
#82468=CARTESIAN_POINT('Ctrl Pts',(18.0929064660597,-20.9709110986508,-14.1501627953669));
#82469=CARTESIAN_POINT('Ctrl Pts',(18.0242288363209,-20.9464708308746,-14.1545393426265));
#82470=CARTESIAN_POINT('Ctrl Pts',(17.9555947609367,-20.922046062761,-14.1589131143435));
#82471=CARTESIAN_POINT('Ctrl Pts',(17.8881727399583,-20.8940565773996,-14.1632868860605));
#82472=CARTESIAN_POINT('Ctrl Pts',(17.8223531243428,-20.8626514528046,-14.1676606577774));
#82473=CARTESIAN_POINT('Ctrl Pts',(17.7565535378573,-20.8312558848945,-14.172033098541));
#82474=CARTESIAN_POINT('Ctrl Pts',(17.6923558237617,-20.7964469488636,-14.1764055393046));
#82475=CARTESIAN_POINT('Ctrl Pts',(17.6301289564777,-20.7584212463523,-14.1807779800681));
#82476=CARTESIAN_POINT('Ctrl Pts',(17.5679004980457,-20.7203945715195,-14.1851505326355));
#82477=CARTESIAN_POINT('Ctrl Pts',(17.5076433970461,-20.6791512201339,-14.1895230852029));
#82478=CARTESIAN_POINT('Ctrl Pts',(17.4496992310181,-20.6349321242381,-14.1938956377702));
#82479=CARTESIAN_POINT('Ctrl Pts',(17.3916949283492,-20.5906671360969,-14.1982727283375));
#82480=CARTESIAN_POINT('Ctrl Pts',(17.3360087376062,-20.5434205306325,-14.2026498189049));
#82481=CARTESIAN_POINT('Ctrl Pts',(17.2829499222238,-20.4934741878428,-14.2070269094722));
#82482=CARTESIAN_POINT('Ctrl Pts',(17.2298621294529,-20.4435005675016,-14.2114063905312));
#82483=CARTESIAN_POINT('Ctrl Pts',(17.1794049028374,-20.3908246228572,-14.2157858715901));
#82484=CARTESIAN_POINT('Ctrl Pts',(17.1318494027602,-20.3357638757259,-14.220165352649));
#82485=CARTESIAN_POINT('Ctrl Pts',(17.0842096108783,-20.2806055337899,-14.2245525963088));
#82486=CARTESIAN_POINT('Ctrl Pts',(17.039482112747,-20.2230543293393,-14.2289398399685));
#82487=CARTESIAN_POINT('Ctrl Pts',(16.9978963120783,-20.1634590314099,-14.2333270836282));
#82488=CARTESIAN_POINT('Ctrl Pts',(16.9696219748223,-20.122939971408,-14.236309986563));
#82489=CARTESIAN_POINT('Ctrl Pts',(16.9427990411454,-20.0814766042669,-14.2392928894977));
#82490=CARTESIAN_POINT('Ctrl Pts',(16.9174873693316,-20.0391848336976,-14.2422757924325));
#82491=CARTESIAN_POINT('Ctrl Pts',(16.8789822269095,-19.9748488759218,-14.2468135054362));
#82492=CARTESIAN_POINT('Ctrl Pts',(16.8438347836027,-19.908358318242,-14.2513512184398));
#82493=CARTESIAN_POINT('Ctrl Pts',(16.8122834229314,-19.8400846791943,-14.2558889314435));
#82494=CARTESIAN_POINT('Ctrl Pts',(16.7877996091002,-19.7871044262843,-14.2594101906868));
#82495=CARTESIAN_POINT('Ctrl Pts',(16.7654805062868,-19.7330511704266,-14.26293144993));
#82496=CARTESIAN_POINT('Ctrl Pts',(16.7454194499637,-19.6781104571739,-14.2664527091733));
#82497=CARTESIAN_POINT('',(16.6170000012625,-18.9520658364028,-13.2889027715975));
#82498=CARTESIAN_POINT('Ctrl Pts',(16.7454194457665,-19.6781104456791,-14.0426552583743));
#82499=CARTESIAN_POINT('Ctrl Pts',(16.7721869599386,-19.7514179686387,-14.0381451037516));
#82500=CARTESIAN_POINT('Ctrl Pts',(16.8029921858641,-19.8232019799891,-14.033765580411));
#82501=CARTESIAN_POINT('Ctrl Pts',(16.8976427025996,-20.0139142964462,-14.0220204986683));
#82502=CARTESIAN_POINT('Ctrl Pts',(16.9689849492002,-20.1286859665614,-14.0148420563074));
#82503=CARTESIAN_POINT('Ctrl Pts',(17.0971457026277,-20.2967112557855,-14.0031497920472));
#82504=CARTESIAN_POINT('Ctrl Pts',(17.1467942036028,-20.3549666617983,-13.9988302072747));
#82505=CARTESIAN_POINT('Ctrl Pts',(17.2060220521686,-20.4172858419015,-13.9937348299809));
#82506=CARTESIAN_POINT('Ctrl Pts',(17.2126111808868,-20.4241261022789,-13.9931687001201));
#82507=CARTESIAN_POINT('Ctrl Pts',(17.2224462448901,-20.4341994572846,-13.9923243406249));
#82508=CARTESIAN_POINT('Ctrl Pts',(17.2256571117406,-20.4374668344645,-13.9920487838485));
#82509=CARTESIAN_POINT('Ctrl Pts',(17.2313903512189,-20.4432632234787,-13.9915568816742));
#82510=CARTESIAN_POINT('Ctrl Pts',(17.2339085440464,-20.445796298648,-13.9913408653148));
#82511=CARTESIAN_POINT('Ctrl Pts',(17.2393381903345,-20.4512304582825,-13.9908751683641));
#82512=CARTESIAN_POINT('Ctrl Pts',(17.2422516423121,-20.4541293982164,-13.9906253322116));
#82513=CARTESIAN_POINT('Ctrl Pts',(17.2503213433811,-20.4621122731473,-13.9899335167327));
#82514=CARTESIAN_POINT('Ctrl Pts',(17.2554952066476,-20.4671782093737,-13.9894901660879));
#82515=CARTESIAN_POINT('Ctrl Pts',(17.2840548107071,-20.4948564945067,-13.987044525901));
#82516=CARTESIAN_POINT('Ctrl Pts',(17.3079320181715,-20.5169527330886,-13.9850059098458));
#82517=CARTESIAN_POINT('Ctrl Pts',(17.4542418792366,-20.6462202684404,-13.9726000407908));
#82518=CARTESIAN_POINT('Ctrl Pts',(17.5881860833947,-20.7395328146315,-13.9616427776728));
#82519=CARTESIAN_POINT('Ctrl Pts',(17.8343782953957,-20.8718996729219,-13.9433846899226));
#82520=CARTESIAN_POINT('Ctrl Pts',(17.9416765416058,-20.9186126484348,-13.93594384611));
#82521=CARTESIAN_POINT('Ctrl Pts',(18.0658261082647,-20.9608396739953,-13.9279367855054));
#82522=CARTESIAN_POINT('Ctrl Pts',(18.0794008270803,-20.9653040316714,-13.9270688094193));
#82523=CARTESIAN_POINT('Ctrl Pts',(18.1010776420677,-20.972190527553,-13.9256945008057));
#82524=CARTESIAN_POINT('Ctrl Pts',(18.1091506623918,-20.9747021004872,-13.9251852402096));
#82525=CARTESIAN_POINT('Ctrl Pts',(18.1234152321935,-20.9790463562849,-13.9242898621162));
#82526=CARTESIAN_POINT('Ctrl Pts',(18.1296004855871,-20.980899188628,-13.9239030884917));
#82527=CARTESIAN_POINT('Ctrl Pts',(18.1424111056422,-20.9846729110359,-13.923105019838));
#82528=CARTESIAN_POINT('Ctrl Pts',(18.1490375853779,-20.9865897764408,-13.9226938601894));
#82529=CARTESIAN_POINT('Ctrl Pts',(18.1660708891544,-20.9914269665598,-13.9216411506931));
#82530=CARTESIAN_POINT('Ctrl Pts',(18.1764910046677,-20.9943000645251,-13.9210011421454));
#82531=CARTESIAN_POINT('Ctrl Pts',(18.2200727018896,-21.0059582694059,-13.9183404789634));
#82532=CARTESIAN_POINT('Ctrl Pts',(18.2534244406701,-21.0140167721381,-13.91634335302));
#82533=CARTESIAN_POINT('Ctrl Pts',(18.3408210802685,-21.0328978569808,-13.9111992821519));
#82534=CARTESIAN_POINT('Ctrl Pts',(18.3951196364458,-21.0424273005058,-13.9080917260888));
#82535=CARTESIAN_POINT('Ctrl Pts',(18.5580873773159,-21.0645104430544,-13.8989473207305));
#82536=CARTESIAN_POINT('Ctrl Pts',(18.6674211618566,-21.0707764782452,-13.8930592008436));
#82537=CARTESIAN_POINT('Ctrl Pts',(18.8224676133939,-21.0676449378191,-13.8846161010564));
#82538=CARTESIAN_POINT('Ctrl Pts',(18.8681428050623,-21.0652405192403,-13.8821158043807));
#82539=CARTESIAN_POINT('Ctrl Pts',(18.9364163957964,-21.059424079672,-13.8783162829452));
#82540=CARTESIAN_POINT('Ctrl Pts',(18.9590966352536,-21.057122348416,-13.8770437146181));
#82541=CARTESIAN_POINT('Ctrl Pts',(18.9827755514586,-21.0543322343119,-13.8757003233075));
#82542=CARTESIAN_POINT('Ctrl Pts',(18.9838163182545,-21.0542088158787,-13.8756412468457));
#82543=CARTESIAN_POINT('Ctrl Pts',(19.0033483655743,-21.051877915128,-13.8745319908282));
#82544=CARTESIAN_POINT('Ctrl Pts',(19.0218093283111,-21.0494273655847,-13.8734739878806));
#82545=CARTESIAN_POINT('Ctrl Pts',(19.0731185568614,-21.0419263239952,-13.8705009022357));
#82546=CARTESIAN_POINT('Ctrl Pts',(19.1058822686279,-21.036345637701,-13.8685651454196));
#82547=CARTESIAN_POINT('Ctrl Pts',(19.1452826450028,-21.028676033506,-13.8661774429272));
#82548=CARTESIAN_POINT('Ctrl Pts',(19.1520597259084,-21.0273223423892,-13.8657645920997));
#82549=CARTESIAN_POINT('Ctrl Pts',(19.1631812398754,-21.0250441846517,-13.8650833640594));
#82550=CARTESIAN_POINT('Ctrl Pts',(19.1675296669947,-21.0241391737013,-13.8648160726923));
#82551=CARTESIAN_POINT('Ctrl Pts',(19.1753596936741,-21.0224838336454,-13.8643330317671));
#82552=CARTESIAN_POINT('Ctrl Pts',(19.1788422714992,-21.021738398384,-13.8641175642141));
#82553=CARTESIAN_POINT('Ctrl Pts',(19.1864403038299,-21.0200919998191,-13.8636460993557));
#82554=CARTESIAN_POINT('Ctrl Pts',(19.1905549045828,-21.0191875499416,-13.8633899088532));
#82555=CARTESIAN_POINT('Ctrl Pts',(19.2021949835671,-21.0165924413463,-13.862662726988));
#82556=CARTESIAN_POINT('Ctrl Pts',(19.2097138695378,-21.0148729484948,-13.8621901298025));
#82557=CARTESIAN_POINT('Ctrl Pts',(19.2565595345929,-21.0038900903622,-13.8592284236552));
#82558=CARTESIAN_POINT('Ctrl Pts',(19.2956210702144,-20.9935441928995,-13.856683039728));
#82559=CARTESIAN_POINT('Ctrl Pts',(19.5037501477926,-20.9319940089521,-13.8427961641896));
#82560=CARTESIAN_POINT('Ctrl Pts',(19.6662060911874,-20.8608973874339,-13.8308635704815));
#82561=CARTESIAN_POINT('Ctrl Pts',(19.8995447047212,-20.7218072092279,-13.813283852132));
#82562=CARTESIAN_POINT('Ctrl Pts',(19.9777804815814,-20.6677291293636,-13.8072854825148));
#82563=CARTESIAN_POINT('Ctrl Pts',(20.0629632242982,-20.599949473611,-13.8006424328673));
#82564=CARTESIAN_POINT('Ctrl Pts',(20.0737134013628,-20.5912219909517,-13.7998017261266));
#82565=CARTESIAN_POINT('Ctrl Pts',(20.0907890903852,-20.5770789752718,-13.7984623470531));
#82566=CARTESIAN_POINT('Ctrl Pts',(20.0971694851617,-20.5717306163295,-13.7979609737402));
#82567=CARTESIAN_POINT('Ctrl Pts',(20.1084262674509,-20.5621810023959,-13.7970747294757));
#82568=CARTESIAN_POINT('Ctrl Pts',(20.1133153272138,-20.5579949111587,-13.7966892445521));
#82569=CARTESIAN_POINT('Ctrl Pts',(20.1234463589306,-20.5492401711612,-13.7958892194195));
#82570=CARTESIAN_POINT('Ctrl Pts',(20.1286850718637,-20.5446678564001,-13.7954748374623));
#82571=CARTESIAN_POINT('Ctrl Pts',(20.1421976389473,-20.5327563778492,-13.7944041255413));
#82572=CARTESIAN_POINT('Ctrl Pts',(20.1504367454304,-20.5253779805447,-13.7937494415916));
#82573=CARTESIAN_POINT('Ctrl Pts',(20.1856586860754,-20.4933346360438,-13.7909422385269));
#82574=CARTESIAN_POINT('Ctrl Pts',(20.2120589428686,-20.4680367406241,-13.7888166847188));
#82575=CARTESIAN_POINT('Ctrl Pts',(20.280153144947,-20.3993153055432,-13.7832614867172));
#82576=CARTESIAN_POINT('Ctrl Pts',(20.3206739306244,-20.3547750297984,-13.7798800177396));
#82577=CARTESIAN_POINT('Ctrl Pts',(20.46575545344,-20.1809590007894,-13.7673401953335));
#82578=CARTESIAN_POINT('Ctrl Pts',(20.5568583641458,-20.0412645572718,-13.7585865664522));
#82579=CARTESIAN_POINT('Ctrl Pts',(20.6550421577045,-19.8432314989794,-13.7461710994383));
#82580=CARTESIAN_POINT('Ctrl Pts',(20.6774818553897,-19.7931740223842,-13.7430275873579));
#82581=CARTESIAN_POINT('Ctrl Pts',(20.7012280681046,-19.7341635254107,-13.7392532697357));
#82582=CARTESIAN_POINT('Ctrl Pts',(20.7044542604594,-19.7260000347712,-13.7387296372469));
#82583=CARTESIAN_POINT('Ctrl Pts',(20.7092558086628,-19.7136256962134,-13.7379333127725));
#82584=CARTESIAN_POINT('Ctrl Pts',(20.7108687182033,-19.7094293900563,-13.7376628193084));
#82585=CARTESIAN_POINT('Ctrl Pts',(20.713736592851,-19.7018964800839,-13.7371763904588));
#82586=CARTESIAN_POINT('Ctrl Pts',(20.7149965068341,-19.6985618176279,-13.736960755355));
#82587=CARTESIAN_POINT('Ctrl Pts',(20.717712138022,-19.6913189744351,-13.7364917291835));
#82588=CARTESIAN_POINT('Ctrl Pts',(20.7191647117576,-19.6874097218526,-13.7362381603033));
#82589=CARTESIAN_POINT('Ctrl Pts',(20.7232031762802,-19.6764420145384,-13.7355256387335));
#82590=CARTESIAN_POINT('Ctrl Pts',(20.725763006085,-19.6693741232079,-13.7350651794537));
#82591=CARTESIAN_POINT('Ctrl Pts',(20.7406603587333,-19.627546914277,-13.7323332428803));
#82592=CARTESIAN_POINT('Ctrl Pts',(20.7521246085084,-19.5924858398115,-13.7300149275892));
#82593=CARTESIAN_POINT('Ctrl Pts',(20.7864934904204,-19.4772689882757,-13.7223447811041));
#82594=CARTESIAN_POINT('Ctrl Pts',(20.8055806134706,-19.3960596634728,-13.7168607867334));
#82595=CARTESIAN_POINT('Ctrl Pts',(20.8507313997309,-19.1358614713703,-13.6994180044698));
#82596=CARTESIAN_POINT('Ctrl Pts',(20.8587061194251,-18.9545165082085,-13.6875290487399));
#82597=CARTESIAN_POINT('Ctrl Pts',(20.8416388849935,-18.7518591691525,-13.6750162408764));
#82598=CARTESIAN_POINT('Ctrl Pts',(20.8393861924423,-18.7294083015744,-13.6736393190221));
#82599=CARTESIAN_POINT('Ctrl Pts',(20.8356783785468,-18.6975854290503,-13.6717001354661));
#82600=CARTESIAN_POINT('Ctrl Pts',(20.834518606021,-18.6881811775329,-13.671128625746));
#82601=CARTESIAN_POINT('Ctrl Pts',(20.832527306908,-18.6728806841485,-13.6702012459747));
#82602=CARTESIAN_POINT('Ctrl Pts',(20.8317339844724,-18.666979681716,-13.6698441748107));
#82603=CARTESIAN_POINT('Ctrl Pts',(20.8300175932237,-18.6546080560707,-13.6690967837867));
#82604=CARTESIAN_POINT('Ctrl Pts',(20.8290894309414,-18.6481381938249,-13.668706629148));
#82605=CARTESIAN_POINT('Ctrl Pts',(20.8268028522558,-18.6327080474139,-13.6677777629402));
#82606=CARTESIAN_POINT('Ctrl Pts',(20.8254168264631,-18.6237519363779,-13.6672399310146));
#82607=CARTESIAN_POINT('Ctrl Pts',(20.8205160816352,-18.5933765669102,-13.6654200705167));
#82608=CARTESIAN_POINT('Ctrl Pts',(20.8167294085277,-18.5720021209686,-13.6641466639462));
#82609=CARTESIAN_POINT('Ctrl Pts',(20.7940292327281,-18.4544251627964,-13.6571759896299));
#82610=CARTESIAN_POINT('Ctrl Pts',(20.7687782534887,-18.359562754452,-13.651686062569));
#82611=CARTESIAN_POINT('Ctrl Pts',(20.6889378443015,-18.1261717353152,-13.6381338850067));
#82612=CARTESIAN_POINT('Ctrl Pts',(20.6261682832087,-17.9910277673772,-13.6302573691986));
#82613=CARTESIAN_POINT('Ctrl Pts',(20.5220671428842,-17.8173596474118,-13.6188753705984));
#82614=CARTESIAN_POINT('Ctrl Pts',(20.4926096792223,-17.7722187550602,-13.6157844445076));
#82615=CARTESIAN_POINT('Ctrl Pts',(20.4564131292788,-17.7211229134234,-13.6120686740366));
#82616=CARTESIAN_POINT('Ctrl Pts',(20.451316812386,-17.7140224759269,-13.6115472680799));
#82617=CARTESIAN_POINT('Ctrl Pts',(20.4435375838022,-17.7033245468187,-13.6107536743237));
#82618=CARTESIAN_POINT('Ctrl Pts',(20.4408868881438,-17.6997035941757,-13.6104836626105));
#82619=CARTESIAN_POINT('Ctrl Pts',(20.4361102326022,-17.6932218384384,-13.6099977473655));
#82620=CARTESIAN_POINT('Ctrl Pts',(20.4339885445472,-17.6903579540658,-13.6097821413715));
#82621=CARTESIAN_POINT('Ctrl Pts',(20.42936489799,-17.6841497302213,-13.6093127659561));
#82622=CARTESIAN_POINT('Ctrl Pts',(20.4268603049836,-17.6808074768039,-13.6090588164771));
#82623=CARTESIAN_POINT('Ctrl Pts',(20.4198030966434,-17.6714478319911,-13.6083441729457));
#82624=CARTESIAN_POINT('Ctrl Pts',(20.4152282293877,-17.6654474078308,-13.6078819581185));
#82625=CARTESIAN_POINT('Ctrl Pts',(20.3878059956778,-17.6298762682055,-13.6051182811268));
#82626=CARTESIAN_POINT('Ctrl Pts',(20.3642124774657,-17.6008921895516,-13.6027687304478));
#82627=CARTESIAN_POINT('Ctrl Pts',(20.2843343202899,-17.5079032402282,-13.5949452046279));
#82628=CARTESIAN_POINT('Ctrl Pts',(20.2249529747154,-17.4466730207191,-13.5893336312393));
#82629=CARTESIAN_POINT('Ctrl Pts',(20.0306366376107,-17.2691124492177,-13.5719446161163));
#82630=CARTESIAN_POINT('Ctrl Pts',(19.8845760090526,-17.1660614841348,-13.5602467270275));
#82631=CARTESIAN_POINT('Ctrl Pts',(19.7071878283161,-17.0718101274938,-13.5478850412963));
#82632=CARTESIAN_POINT('Ctrl Pts',(19.6868879283737,-17.0614410441462,-13.5464938043774));
#82633=CARTESIAN_POINT('Ctrl Pts',(19.65788285135,-17.0472113020174,-13.5445381840105));
#82634=CARTESIAN_POINT('Ctrl Pts',(19.6493135602774,-17.0430786820891,-13.5439643377366));
#82635=CARTESIAN_POINT('Ctrl Pts',(19.635330110926,-17.0364508454563,-13.5430342102175));
#82636=CARTESIAN_POINT('Ctrl Pts',(19.629932829043,-17.0339205179901,-13.5426767135916));
#82637=CARTESIAN_POINT('Ctrl Pts',(19.6186009854747,-17.0286662448261,-13.5419292622041));
#82638=CARTESIAN_POINT('Ctrl Pts',(19.6126643554615,-17.025946888269,-13.541539469021));
#82639=CARTESIAN_POINT('Ctrl Pts',(19.598489721046,-17.0195331742507,-13.5406129797373));
#82640=CARTESIAN_POINT('Ctrl Pts',(19.5902404356889,-17.0158639431713,-13.5400771513667));
#82641=CARTESIAN_POINT('Ctrl Pts',(19.5622666238311,-17.0036351185028,-13.5382712670726));
#82642=CARTESIAN_POINT('Ctrl Pts',(19.542434844009,-16.9953231067151,-13.5370096516184));
#82643=CARTESIAN_POINT('Ctrl Pts',(19.3557094266094,-16.9203853492735,-13.5252950445415));
#82644=CARTESIAN_POINT('Ctrl Pts',(19.1810999362263,-16.8749614081036,-13.5156412900567));
#82645=CARTESIAN_POINT('Ctrl Pts',(18.8835838187848,-16.8368716329855,-13.4993166157163));
#82646=CARTESIAN_POINT('Ctrl Pts',(18.7632637349034,-16.8317928083396,-13.4927195868004));
#82647=CARTESIAN_POINT('Ctrl Pts',(18.6336873316197,-16.8373566003335,-13.4850331194839));
#82648=CARTESIAN_POINT('Ctrl Pts',(18.6241944420691,-16.8378282777837,-13.4844665819589));
#82649=CARTESIAN_POINT('Ctrl Pts',(18.6101301512917,-16.8386220738344,-13.4836217296178));
#82650=CARTESIAN_POINT('Ctrl Pts',(18.6055559505523,-16.8388951461229,-13.4833460921917));
#82651=CARTESIAN_POINT('Ctrl Pts',(18.5974177730034,-16.8394075039179,-13.4828541018001));
#82652=CARTESIAN_POINT('Ctrl Pts',(18.5938534796924,-16.8396409604782,-13.4826380783304));
#82653=CARTESIAN_POINT('Ctrl Pts',(18.5861900995733,-16.8401623835543,-13.4821724296963));
#82654=CARTESIAN_POINT('Ctrl Pts',(18.5820913155066,-16.8404532598564,-13.4819226493064));
#82655=CARTESIAN_POINT('Ctrl Pts',(18.5707761194048,-16.8412893758241,-13.4812311418009));
#82656=CARTESIAN_POINT('Ctrl Pts',(18.5635616956397,-16.8418596835451,-13.4807880453361));
#82657=CARTESIAN_POINT('Ctrl Pts',(18.523994794911,-16.8451917203648,-13.4783463696751));
#82658=CARTESIAN_POINT('Ctrl Pts',(18.4917080993436,-16.8486603506387,-13.4763115998307));
#82659=CARTESIAN_POINT('Ctrl Pts',(18.2981304459386,-16.8739727174034,-13.4639070236209));
#82660=CARTESIAN_POINT('Ctrl Pts',(18.13972130921,-16.9136152437953,-13.4529462357759));
#82661=CARTESIAN_POINT('Ctrl Pts',(17.8781151470345,-17.0122076422301,-13.4346849232696));
#82662=CARTESIAN_POINT('Ctrl Pts',(17.7723945378792,-17.062382045708,-13.4272441800145));
#82663=CARTESIAN_POINT('Ctrl Pts',(17.6578777315532,-17.1288455590383,-13.4191593261585));
#82664=CARTESIAN_POINT('Ctrl Pts',(17.6445025247068,-17.1368067530198,-13.4182143261785));
#82665=CARTESIAN_POINT('Ctrl Pts',(17.6244411519992,-17.1490493197416,-13.4167955644284));
#82666=CARTESIAN_POINT('Ctrl Pts',(17.6176894899693,-17.153221847894,-13.4163178422648));
#82667=CARTESIAN_POINT('Ctrl Pts',(17.6057065981157,-17.1607207292496,-13.415469498479));
#82668=CARTESIAN_POINT('Ctrl Pts',(17.6004662421755,-17.164032257647,-13.4150983360449));
#82669=CARTESIAN_POINT('Ctrl Pts',(17.5902140547062,-17.1705740927647,-13.4143718399567));
#82670=CARTESIAN_POINT('Ctrl Pts',(17.5852011793017,-17.1738026481008,-13.4140164459822));
#82671=CARTESIAN_POINT('Ctrl Pts',(17.5714896433962,-17.1827157804008,-13.4130438407229));
#82672=CARTESIAN_POINT('Ctrl Pts',(17.562819017157,-17.1884433408034,-13.4124282396084));
#82673=CARTESIAN_POINT('Ctrl Pts',(17.5285817782131,-17.2114233183363,-13.4099948154214));
#82674=CARTESIAN_POINT('Ctrl Pts',(17.5033505548447,-17.2291702459126,-13.4081956962966));
#82675=CARTESIAN_POINT('Ctrl Pts',(17.4401260604431,-17.2757385457438,-13.4036643613956));
#82676=CARTESIAN_POINT('Ctrl Pts',(17.402701510518,-17.3053042146353,-13.4009603597374));
#82677=CARTESIAN_POINT('Ctrl Pts',(17.2129193101145,-17.465936499037,-13.3870466588676));
#82678=CARTESIAN_POINT('Ctrl Pts',(17.0788208989739,-17.6169206488171,-13.3766113981987));
#82679=CARTESIAN_POINT('Ctrl Pts',(16.9454163218237,-17.81871376139,-13.3628534654534));
#82680=CARTESIAN_POINT('Ctrl Pts',(16.9238101457127,-17.853554977078,-13.3604799994511));
#82681=CARTESIAN_POINT('Ctrl Pts',(16.8995229162862,-17.8953840110384,-13.3576059848227));
#82682=CARTESIAN_POINT('Ctrl Pts',(16.8958488670851,-17.9017886271043,-13.3571652684421));
#82683=CARTESIAN_POINT('Ctrl Pts',(16.8899474763337,-17.9122017894717,-13.3564474244174));
#82684=CARTESIAN_POINT('Ctrl Pts',(16.8876994874731,-17.9161986458817,-13.3561715901209));
#82685=CARTESIAN_POINT('Ctrl Pts',(16.8837234237483,-17.9233220363606,-13.3556793842589));
#82686=CARTESIAN_POINT('Ctrl Pts',(16.8819902588821,-17.9264456718049,-13.355463343305));
#82687=CARTESIAN_POINT('Ctrl Pts',(16.8782815021483,-17.9331699240814,-13.3549978120319));
#82688=CARTESIAN_POINT('Ctrl Pts',(16.8763085082727,-17.9367718543269,-13.354748167305));
#82689=CARTESIAN_POINT('Ctrl Pts',(16.870892553817,-17.9467279602914,-13.3540574089041));
#82690=CARTESIAN_POINT('Ctrl Pts',(16.8674716687201,-17.9530939909571,-13.3536149306657));
#82691=CARTESIAN_POINT('Ctrl Pts',(16.8489285518339,-17.9880292930581,-13.3511828650674));
#82692=CARTESIAN_POINT('Ctrl Pts',(16.834430467357,-18.0169228828917,-13.3491574153013));
#82693=CARTESIAN_POINT('Ctrl Pts',(16.7509029235034,-18.1933526890104,-13.3367559519128));
#82694=CARTESIAN_POINT('Ctrl Pts',(16.6984298740533,-18.3481176259676,-13.3257865964695));
#82695=CARTESIAN_POINT('Ctrl Pts',(16.6510960514021,-18.5684579652946,-13.3110654529574));
#82696=CARTESIAN_POINT('Ctrl Pts',(16.6406827342214,-18.6301037482727,-13.3070327355362));
#82697=CARTESIAN_POINT('Ctrl Pts',(16.6297590815427,-18.7184169347304,-13.3013962992466));
#82698=CARTESIAN_POINT('Ctrl Pts',(16.6270006057081,-18.7447693600014,-13.2997318572692));
#82699=CARTESIAN_POINT('Ctrl Pts',(16.6216845006033,-18.8067773718103,-13.2958565756987));
#82700=CARTESIAN_POINT('Ctrl Pts',(16.6195337088767,-18.8424603781411,-13.2936584428369));
#82701=CARTESIAN_POINT('Ctrl Pts',(16.6178981528545,-18.8893377127938,-13.2908108214091));
#82702=CARTESIAN_POINT('Ctrl Pts',(16.6175971716164,-18.9004959689164,-13.2901359625467));
#82703=CARTESIAN_POINT('Ctrl Pts',(16.6172522422916,-18.9185925226664,-13.2890461501006));
#82704=CARTESIAN_POINT('Ctrl Pts',(16.6171541289577,-18.9255294627886,-13.288629507179));
#82705=CARTESIAN_POINT('Ctrl Pts',(16.6170502015161,-18.9367926100214,-13.2879547992264));
#82706=CARTESIAN_POINT('Ctrl Pts',(16.6170235456918,-18.9411185320172,-13.2876960836696));
#82707=CARTESIAN_POINT('Ctrl Pts',(16.6170034293768,-18.9476147918886,-13.2873081980846));
#82708=CARTESIAN_POINT('Ctrl Pts',(16.6170000462454,-18.9497850674194,-13.2871787183687));
#82709=CARTESIAN_POINT('Ctrl Pts',(16.6170000004709,-18.9519553492827,-13.287049342907));
#82710=CARTESIAN_POINT('Ctrl Pts',(16.6170000013281,-18.9520749873283,-13.2890562789747));
#82711=CARTESIAN_POINT('Ctrl Pts',(16.6170027225446,-19.0288988399567,-13.2844612169082));
#82712=CARTESIAN_POINT('Ctrl Pts',(16.6211915380442,-19.1056371710189,-13.2798661548417));
#82713=CARTESIAN_POINT('Ctrl Pts',(16.6295128869012,-19.1818325277265,-13.2752710927752));
#82714=CARTESIAN_POINT('Ctrl Pts',(16.6378461991752,-19.2581374287929,-13.2706694244908));
#82715=CARTESIAN_POINT('Ctrl Pts',(16.6503238258348,-19.3338973983149,-13.2660677562064));
#82716=CARTESIAN_POINT('Ctrl Pts',(16.6668410730001,-19.4086650528829,-13.261466087922));
#82717=CARTESIAN_POINT('Ctrl Pts',(16.6833972601622,-19.4836089748522,-13.2568535710412));
#82718=CARTESIAN_POINT('Ctrl Pts',(16.7040119873824,-19.5575555160791,-13.2522410541604));
#82719=CARTESIAN_POINT('Ctrl Pts',(16.7285306582113,-19.6300720604371,-13.2476285372796));
#82720=CARTESIAN_POINT('Ctrl Pts',(16.7339690427624,-19.6461566539819,-13.2466054540659));
#82721=CARTESIAN_POINT('Ctrl Pts',(16.739599307015,-19.662170977234,-13.2455823708523));
#82722=CARTESIAN_POINT('Ctrl Pts',(16.7454194499637,-19.6781104571739,-13.2445592876386));
#82723=CARTESIAN_POINT('Origin',(18.734,-18.952,0.));
#82724=CARTESIAN_POINT('',(16.7437496527793,-19.6787359237804,-12.4443820746906));
#82725=CARTESIAN_POINT('',(16.7454195349593,-19.6781106899492,-12.6679318731853));
#82726=CARTESIAN_POINT('',(16.7454194499637,-19.6781104571739,0.));
#82727=CARTESIAN_POINT('Ctrl Pts',(16.7454195349593,-19.6781106899492,-12.6679318731853));
#82728=CARTESIAN_POINT('Ctrl Pts',(16.705203908673,-19.5679731999918,-12.6745735390896));
#82729=CARTESIAN_POINT('Ctrl Pts',(16.6741842980992,-19.4546217778048,-12.6809438288943));
#82730=CARTESIAN_POINT('Ctrl Pts',(16.6289120093902,-19.2112807481602,-12.6943852262644));
#82731=CARTESIAN_POINT('Ctrl Pts',(16.6169601911292,-19.0814434066492,-12.7014276312587));
#82732=CARTESIAN_POINT('Ctrl Pts',(16.6170011043058,-18.9480754918077,-12.7092186189957));
#82733=CARTESIAN_POINT('Ctrl Pts',(16.6170097089921,-18.9448004415573,-12.7094102891661));
#82734=CARTESIAN_POINT('Ctrl Pts',(16.6171033910119,-18.9258667099555,-12.7105204682452));
#82735=CARTESIAN_POINT('Ctrl Pts',(16.6173545994999,-18.9102098313582,-12.7114467924583));
#82736=CARTESIAN_POINT('Ctrl Pts',(16.6179364418611,-18.8887742899,-12.7127280957681));
#82737=CARTESIAN_POINT('Ctrl Pts',(16.6181171311767,-18.8829916227347,-12.7130750584379));
#82738=CARTESIAN_POINT('Ctrl Pts',(16.6184419953724,-18.873801800889,-12.7136286293193));
#82739=CARTESIAN_POINT('Ctrl Pts',(16.6185707048855,-18.8703940793869,-12.713834377607));
#82740=CARTESIAN_POINT('Ctrl Pts',(16.6188536040123,-18.8633550108911,-12.7142603867494));
#82741=CARTESIAN_POINT('Ctrl Pts',(16.6190089114769,-18.8597237558016,-12.7144807118296));
#82742=CARTESIAN_POINT('Ctrl Pts',(16.619401390337,-18.851069284925,-12.7150071270833));
#82743=CARTESIAN_POINT('Ctrl Pts',(16.6196471101571,-18.8460464948671,-12.7153136921317));
#82744=CARTESIAN_POINT('Ctrl Pts',(16.6205368798928,-18.8290963045789,-12.7163516784865));
#82745=CARTESIAN_POINT('Ctrl Pts',(16.6212639670735,-18.8171737470573,-12.7170875273693));
#82746=CARTESIAN_POINT('Ctrl Pts',(16.6311147089677,-18.6754017636838,-12.7259008176317));
#82747=CARTESIAN_POINT('Ctrl Pts',(16.6520942072658,-18.546667431601,-12.7345184188496));
#82748=CARTESIAN_POINT('Ctrl Pts',(16.7254963566545,-18.2635581636166,-12.7538450628526));
#82749=CARTESIAN_POINT('Ctrl Pts',(16.7841810481341,-18.1116049299082,-12.7644509320186));
#82750=CARTESIAN_POINT('Ctrl Pts',(16.870698255241,-17.9468342438934,-12.7759141291557));
#82751=CARTESIAN_POINT('Ctrl Pts',(16.8820773745263,-17.926020346037,-12.7773627665996));
#82752=CARTESIAN_POINT('Ctrl Pts',(16.8985833941536,-17.8969984203578,-12.7793842792735));
#82753=CARTESIAN_POINT('Ctrl Pts',(16.903420087807,-17.8886281741606,-12.7799675007672));
#82754=CARTESIAN_POINT('Ctrl Pts',(16.9113458117626,-17.875126480648,-12.7809086731479));
#82755=CARTESIAN_POINT('Ctrl Pts',(16.9143995407292,-17.8699745676057,-12.781267897193));
#82756=CARTESIAN_POINT('Ctrl Pts',(16.9208163406894,-17.8592528430474,-12.7820157145292));
#82757=CARTESIAN_POINT('Ctrl Pts',(16.9241833133214,-17.8536854305361,-12.7824041604479));
#82758=CARTESIAN_POINT('Ctrl Pts',(16.9322154953229,-17.8405411526983,-12.7833216135196));
#82759=CARTESIAN_POINT('Ctrl Pts',(16.9369029358397,-17.8329779643774,-12.7838497980817));
#82760=CARTESIAN_POINT('Ctrl Pts',(16.9526722795969,-17.8078887681429,-12.7856030771217));
#82761=CARTESIAN_POINT('Ctrl Pts',(16.9639641920581,-17.7904956986808,-12.7868203958941));
#82762=CARTESIAN_POINT('Ctrl Pts',(17.0256057783288,-17.6985355508069,-12.7932713109868));
#82763=CARTESIAN_POINT('Ctrl Pts',(17.0804177574797,-17.6270651376852,-12.7983319640066));
#82764=CARTESIAN_POINT('Ctrl Pts',(17.2287617866374,-17.4572396203864,-12.8107688205488));
#82765=CARTESIAN_POINT('Ctrl Pts',(17.3274941930707,-17.3639855649346,-12.8179810344386));
#82766=CARTESIAN_POINT('Ctrl Pts',(17.4939762702954,-17.2345266456223,-12.8296568863137));
#82767=CARTESIAN_POINT('Ctrl Pts',(17.5559186344873,-17.191461641878,-12.8339175550008));
#82768=CARTESIAN_POINT('Ctrl Pts',(17.628087431752,-17.14680293386,-12.8389474843062));
#82769=CARTESIAN_POINT('Ctrl Pts',(17.6361904509646,-17.1418637502464,-12.8395131452152));
#82770=CARTESIAN_POINT('Ctrl Pts',(17.6482524532083,-17.1346221537431,-12.840356937765));
#82771=CARTESIAN_POINT('Ctrl Pts',(17.6521862699813,-17.1322777618361,-12.8406324017569));
#82772=CARTESIAN_POINT('Ctrl Pts',(17.659201726931,-17.1281276279674,-12.8411242025125));
#82773=CARTESIAN_POINT('Ctrl Pts',(17.6622803605305,-17.1263169028005,-12.8413402107637));
#82774=CARTESIAN_POINT('Ctrl Pts',(17.6689124561005,-17.1224387343665,-12.8418059635862));
#82775=CARTESIAN_POINT('Ctrl Pts',(17.6724673101804,-17.1203738785831,-12.8420558641062));
#82776=CARTESIAN_POINT('Ctrl Pts',(17.682304247197,-17.1146982975689,-12.8427480350089));
#82777=CARTESIAN_POINT('Ctrl Pts',(17.6885988189649,-17.111109490107,-12.8431916789839));
#82778=CARTESIAN_POINT('Ctrl Pts',(17.7233141666129,-17.0915522363204,-12.8456419033174));
#82779=CARTESIAN_POINT('Ctrl Pts',(17.7520807967276,-17.0762105281185,-12.8476849676134));
#82780=CARTESIAN_POINT('Ctrl Pts',(17.9264334001353,-16.9883349739594,-12.8600923397222));
#82781=CARTESIAN_POINT('Ctrl Pts',(18.0796267753151,-16.9321139217962,-12.8710455363536));
#82782=CARTESIAN_POINT('Ctrl Pts',(18.3512832304712,-16.8666085870997,-12.8892984222841));
#82783=CARTESIAN_POINT('Ctrl Pts',(18.466906264726,-16.8486697335391,-12.8967379837458));
#82784=CARTESIAN_POINT('Ctrl Pts',(18.5976891560913,-16.8393446726929,-12.9047438507408));
#82785=CARTESIAN_POINT('Ctrl Pts',(18.6119522531885,-16.8384727251865,-12.9056118112131));
#82786=CARTESIAN_POINT('Ctrl Pts',(18.6346668420434,-16.8373148221815,-12.9069860999014));
#82787=CARTESIAN_POINT('Ctrl Pts',(18.6431129150329,-16.8369349847864,-12.9074953560532));
#82788=CARTESIAN_POINT('Ctrl Pts',(18.6580129430798,-16.8363543169417,-12.9083907290304));
#82789=CARTESIAN_POINT('Ctrl Pts',(18.6644659235801,-16.8361323995316,-12.9087775019588));
#82790=CARTESIAN_POINT('Ctrl Pts',(18.6778148994949,-16.8357344641797,-12.9095755717601));
#82791=CARTESIAN_POINT('Ctrl Pts',(18.684710949815,-16.8355626220266,-12.9099867332395));
#82792=CARTESIAN_POINT('Ctrl Pts',(18.7024144005585,-16.8352080452256,-12.9110394527732));
#82793=CARTESIAN_POINT('Ctrl Pts',(18.7132226678653,-16.8350743662287,-12.9116794694701));
#82794=CARTESIAN_POINT('Ctrl Pts',(18.7583375662738,-16.8348619304341,-12.9143402112538));
#82795=CARTESIAN_POINT('Ctrl Pts',(18.7926436655862,-16.8355343045908,-12.916337405879));
#82796=CARTESIAN_POINT('Ctrl Pts',(18.8819742592859,-16.8394590026465,-12.9214816934866));
#82797=CARTESIAN_POINT('Ctrl Pts',(18.9369158048235,-16.8440266442537,-12.9245893932608));
#82798=CARTESIAN_POINT('Ctrl Pts',(19.1001555303925,-16.8640401745045,-12.933734049447));
#82799=CARTESIAN_POINT('Ctrl Pts',(19.2075002585101,-16.8857365865225,-12.9396222772934));
#82800=CARTESIAN_POINT('Ctrl Pts',(19.3568799015149,-16.9281867031771,-12.9480771552648));
#82801=CARTESIAN_POINT('Ctrl Pts',(19.4006500509014,-16.9421798337911,-12.9505892003355));
#82802=CARTESIAN_POINT('Ctrl Pts',(19.4649308619058,-16.9650611373605,-12.9543731912886));
#82803=CARTESIAN_POINT('Ctrl Pts',(19.4858128918095,-16.9728680448278,-12.9556176889191));
#82804=CARTESIAN_POINT('Ctrl Pts',(19.5544199653136,-16.9997598042307,-12.9597686828353));
#82805=CARTESIAN_POINT('Ctrl Pts',(19.6015696907667,-17.0202514108216,-12.962722046598));
#82806=CARTESIAN_POINT('Ctrl Pts',(19.655028173563,-17.0458367978539,-12.966239644708));
#82807=CARTESIAN_POINT('Ctrl Pts',(19.662114325814,-17.0492769924216,-12.9667094238342));
#82808=CARTESIAN_POINT('Ctrl Pts',(19.6733817024066,-17.0548250103043,-12.9674622631931));
#82809=CARTESIAN_POINT('Ctrl Pts',(19.6775754958605,-17.0569073355133,-12.9677437783263));
#82810=CARTESIAN_POINT('Ctrl Pts',(19.6849751951,-17.0606121263562,-12.9682428623996));
#82811=CARTESIAN_POINT('Ctrl Pts',(19.6881839214519,-17.0622288619646,-12.9684600714186));
#82812=CARTESIAN_POINT('Ctrl Pts',(19.6949590056986,-17.065664182877,-12.9689203964719));
#82813=CARTESIAN_POINT('Ctrl Pts',(19.6985242700208,-17.0674846889663,-12.9691636273886));
#82814=CARTESIAN_POINT('Ctrl Pts',(19.7080948112366,-17.0724059010699,-12.9698191827902));
#82815=CARTESIAN_POINT('Ctrl Pts',(19.7140903794447,-17.0755252404361,-12.9702326551764));
#82816=CARTESIAN_POINT('Ctrl Pts',(19.7432952134849,-17.0908979102039,-12.972259997549));
#82817=CARTESIAN_POINT('Ctrl Pts',(19.7662890636642,-17.1035528249061,-12.9738973123395));
#82818=CARTESIAN_POINT('Ctrl Pts',(19.831477636975,-17.1410257200416,-12.9786454183624));
#82819=CARTESIAN_POINT('Ctrl Pts',(19.8730532935303,-17.1668832060134,-12.9818037835828));
#82820=CARTESIAN_POINT('Ctrl Pts',(19.993943561746,-17.2480129179584,-12.9913042266508));
#82821=CARTESIAN_POINT('Ctrl Pts',(20.0704112864608,-17.3073011131475,-12.9977331014421));
#82822=CARTESIAN_POINT('Ctrl Pts',(20.2478325446529,-17.4654316091008,-13.0133685743738));
#82823=CARTESIAN_POINT('Ctrl Pts',(20.3434827441866,-17.5695553533997,-13.0224360878211));
#82824=CARTESIAN_POINT('Ctrl Pts',(20.4366434862985,-17.6938671981591,-13.0319214172026));
#82825=CARTESIAN_POINT('Ctrl Pts',(20.4450929332443,-17.70538298664,-13.0327889690181));
#82826=CARTESIAN_POINT('Ctrl Pts',(20.4583563904069,-17.7238487536606,-13.0341627349987));
#82827=CARTESIAN_POINT('Ctrl Pts',(20.4632463177956,-17.730743425545,-13.0346718736355));
#82828=CARTESIAN_POINT('Ctrl Pts',(20.4717983283495,-17.7429558920469,-13.0355671099326));
#82829=CARTESIAN_POINT('Ctrl Pts',(20.4754775983943,-17.7482614649711,-13.0359538630655));
#82830=CARTESIAN_POINT('Ctrl Pts',(20.4830379644293,-17.7592708633556,-13.0367519590075));
#82831=CARTESIAN_POINT('Ctrl Pts',(20.4869155702732,-17.7649770012162,-13.037163166093));
#82832=CARTESIAN_POINT('Ctrl Pts',(20.4967986024945,-17.7796745358065,-13.0382161410989));
#82833=CARTESIAN_POINT('Ctrl Pts',(20.5027632109011,-17.7886932402494,-13.0388563661931));
#82834=CARTESIAN_POINT('Ctrl Pts',(20.5273801485272,-17.8265420060082,-13.0415191343029));
#82835=CARTESIAN_POINT('Ctrl Pts',(20.5453993771964,-17.8557789699148,-13.0435181010877));
#82836=CARTESIAN_POINT('Ctrl Pts',(20.5904983054417,-17.9331047852169,-13.0486679860457));
#82837=CARTESIAN_POINT('Ctrl Pts',(20.6164237228005,-17.9818376464868,-13.0517793984954));
#82838=CARTESIAN_POINT('Ctrl Pts',(20.6879862345602,-18.1300533123686,-13.0609305311442));
#82839=CARTESIAN_POINT('Ctrl Pts',(20.727847880218,-18.2321180169854,-13.0668215445066));
#82840=CARTESIAN_POINT('Ctrl Pts',(20.7744330181973,-18.3855083481516,-13.0755497076273));
#82841=CARTESIAN_POINT('Ctrl Pts',(20.7874623617863,-18.4347266943472,-13.0783341369971));
#82842=CARTESIAN_POINT('Ctrl Pts',(20.8021800539444,-18.4997083215456,-13.0820409998631));
#82843=CARTESIAN_POINT('Ctrl Pts',(20.8054839908773,-18.5150897620407,-13.0829206782023));
#82844=CARTESIAN_POINT('Ctrl Pts',(20.8191178946672,-18.5821966201499,-13.0867737076442));
#82845=CARTESIAN_POINT('Ctrl Pts',(20.8276832347021,-18.6342568668373,-13.08980165725));
#82846=CARTESIAN_POINT('Ctrl Pts',(20.8353850232781,-18.695201363867,-13.0934472532827));
#82847=CARTESIAN_POINT('Ctrl Pts',(20.8364216869795,-18.7038315091866,-13.0939658392605));
#82848=CARTESIAN_POINT('Ctrl Pts',(20.8379117367722,-18.716916080413,-13.0947559733477));
#82849=CARTESIAN_POINT('Ctrl Pts',(20.8384042010401,-18.7213660840759,-13.0950253736331));
#82850=CARTESIAN_POINT('Ctrl Pts',(20.8392632774873,-18.7293607590349,-13.0955106389907));
#82851=CARTESIAN_POINT('Ctrl Pts',(20.8396350588734,-18.7329048204634,-13.0957262100106));
#82852=CARTESIAN_POINT('Ctrl Pts',(20.8404239568868,-18.7406126208114,-13.0961960375615));
#82853=CARTESIAN_POINT('Ctrl Pts',(20.8408376718702,-18.744776608666,-13.0964504770346));
#82854=CARTESIAN_POINT('Ctrl Pts',(20.8419662927908,-18.7564888838651,-13.0971678554369));
#82855=CARTESIAN_POINT('Ctrl Pts',(20.8426529878658,-18.7640397359935,-13.097632333511));
#82856=CARTESIAN_POINT('Ctrl Pts',(20.8465378410405,-18.8094612654796,-13.100437644118));
#82857=CARTESIAN_POINT('Ctrl Pts',(20.8487560509632,-18.8474062613524,-13.1028282312516));
#82858=CARTESIAN_POINT('Ctrl Pts',(20.8527120532288,-18.9730690375215,-13.1108564341275));
#82859=CARTESIAN_POINT('Ctrl Pts',(20.8500194555176,-19.0608319706576,-13.1166390368668));
#82860=CARTESIAN_POINT('Ctrl Pts',(20.8257290822401,-19.3218395735466,-13.1339593892005));
#82861=CARTESIAN_POINT('Ctrl Pts',(20.7881616401392,-19.4928834194246,-13.1454065362316));
#82862=CARTESIAN_POINT('Ctrl Pts',(20.7223354015534,-19.6791474167087,-13.1575672063208));
#82863=CARTESIAN_POINT('Ctrl Pts',(20.7142945423085,-19.7007687403044,-13.1589753661778));
#82864=CARTESIAN_POINT('Ctrl Pts',(20.7024239030545,-19.7311583289424,-13.1609503969806));
#82865=CARTESIAN_POINT('Ctrl Pts',(20.6988858337083,-19.7400380884553,-13.1615269876774));
#82866=CARTESIAN_POINT('Ctrl Pts',(20.6930408000488,-19.7544236867725,-13.1624603452406));
#82867=CARTESIAN_POINT('Ctrl Pts',(20.690770505534,-19.7599441930948,-13.1628183443127));
#82868=CARTESIAN_POINT('Ctrl Pts',(20.6859705830224,-19.7714768983658,-13.1635658828843));
#82869=CARTESIAN_POINT('Ctrl Pts',(20.6834364534085,-19.7774871649704,-13.1639552650303));
#82870=CARTESIAN_POINT('Ctrl Pts',(20.6773439872508,-19.791752314378,-13.1648790281169));
#82871=CARTESIAN_POINT('Ctrl Pts',(20.6737607535061,-19.799996477139,-13.1654125549704));
#82872=CARTESIAN_POINT('Ctrl Pts',(20.6615229563997,-19.8276692370202,-13.1672024814055));
#82873=CARTESIAN_POINT('Ctrl Pts',(20.6526279719372,-19.8469905664031,-13.1684506452609));
#82874=CARTESIAN_POINT('Ctrl Pts',(20.5767438129362,-20.0054902695259,-13.1786845902747));
#82875=CARTESIAN_POINT('Ctrl Pts',(20.4949977213949,-20.1370911318832,-13.1871018764965));
#82876=CARTESIAN_POINT('Ctrl Pts',(20.3152312142637,-20.3662502057235,-13.2029185793079));
#82877=CARTESIAN_POINT('Ctrl Pts',(20.2205947451412,-20.4654138490875,-13.2103041963936));
#82878=CARTESIAN_POINT('Ctrl Pts',(20.1052748682238,-20.5649281362042,-13.2192364240755));
#82879=CARTESIAN_POINT('Ctrl Pts',(20.0933629325293,-20.5749800745963,-13.2201585288741));
#82880=CARTESIAN_POINT('Ctrl Pts',(20.0768874313485,-20.5885743771724,-13.2214348812018));
#82881=CARTESIAN_POINT('Ctrl Pts',(20.0724184152457,-20.5922312304195,-13.2217811920167));
#82882=CARTESIAN_POINT('Ctrl Pts',(20.0652881973517,-20.5980171172175,-13.222333979641));
#82883=CARTESIAN_POINT('Ctrl Pts',(20.0626366811656,-20.6001581185257,-13.2225396008818));
#82884=CARTESIAN_POINT('Ctrl Pts',(20.057145599092,-20.6045701026581,-13.2229655689635));
#82885=CARTESIAN_POINT('Ctrl Pts',(20.0543053566104,-20.6068401690569,-13.2231859810243));
#82886=CARTESIAN_POINT('Ctrl Pts',(20.0475167370122,-20.6122373777806,-13.2237129696987));
#82887=CARTESIAN_POINT('Ctrl Pts',(20.0435630325112,-20.6153577581711,-13.2240200239175));
#82888=CARTESIAN_POINT('Ctrl Pts',(20.0301588734137,-20.6258593036124,-13.2250613688593));
#82889=CARTESIAN_POINT('Ctrl Pts',(20.0206570535133,-20.633174114956,-13.2258001254407));
#82890=CARTESIAN_POINT('Ctrl Pts',(19.9093804162313,-20.7173425996273,-13.2344534122617));
#82891=CARTESIAN_POINT('Ctrl Pts',(19.8009334406734,-20.7849211402687,-13.242886937252));
#82892=CARTESIAN_POINT('Ctrl Pts',(19.5396963320284,-20.9166338298046,-13.262220692687));
#82893=CARTESIAN_POINT('Ctrl Pts',(19.3841004551618,-20.9734652468898,-13.2730159395898));
#82894=CARTESIAN_POINT('Ctrl Pts',(19.20049174163,-21.0170984707196,-13.2846391271698));
#82895=CARTESIAN_POINT('Ctrl Pts',(19.1774350585562,-21.0221718910315,-13.286080754895));
#82896=CARTESIAN_POINT('Ctrl Pts',(19.1448415986351,-21.0287742452012,-13.288094211721));
#82897=CARTESIAN_POINT('Ctrl Pts',(19.1353725087011,-21.0306250741248,-13.2886762773883));
#82898=CARTESIAN_POINT('Ctrl Pts',(19.1200090256569,-21.0335191224342,-13.2896160865066));
#82899=CARTESIAN_POINT('Ctrl Pts',(19.1141223600509,-21.0346021745597,-13.2899750959463));
#82900=CARTESIAN_POINT('Ctrl Pts',(19.101824633021,-21.0368108802772,-13.2907228579707));
#82901=CARTESIAN_POINT('Ctrl Pts',(19.0954128061921,-21.0379319624952,-13.2911114614653));
#82902=CARTESIAN_POINT('Ctrl Pts',(19.0802087498384,-21.0405181226784,-13.2920299871718));
#82903=CARTESIAN_POINT('Ctrl Pts',(19.0714121924375,-21.0419572874384,-13.2925590814457));
#82904=CARTESIAN_POINT('Ctrl Pts',(19.0426192480071,-21.0464814445051,-13.2942834838662));
#82905=CARTESIAN_POINT('Ctrl Pts',(19.0225873094142,-21.0493353971963,-13.2954714804212));
#82906=CARTESIAN_POINT('Ctrl Pts',(18.9749216392829,-21.0554304646181,-13.2982724891217));
#82907=CARTESIAN_POINT('Ctrl Pts',(18.947258561768,-21.0584149263371,-13.2998775423216));
#82908=CARTESIAN_POINT('Ctrl Pts',(18.750836523532,-21.0756967747023,-13.3111481661307));
#82909=CARTESIAN_POINT('Ctrl Pts',(18.5809630246235,-21.0702430855674,-13.320175318181));
#82910=CARTESIAN_POINT('Ctrl Pts',(18.3107914109264,-21.028870241372,-13.3351121817024));
#82911=CARTESIAN_POINT('Ctrl Pts',(18.2093467407402,-21.0055892059446,-13.3408765441184));
#82912=CARTESIAN_POINT('Ctrl Pts',(18.100779628979,-20.9721026746093,-13.3476075994602));
#82913=CARTESIAN_POINT('Ctrl Pts',(18.091542052835,-20.9691838370138,-13.3481849116236));
#82914=CARTESIAN_POINT('Ctrl Pts',(18.0779311492103,-20.9647801643989,-13.3490427800663));
#82915=CARTESIAN_POINT('Ctrl Pts',(18.0735419745929,-20.9633442079671,-13.3493205378534));
#82916=CARTESIAN_POINT('Ctrl Pts',(18.0657629024586,-20.96077100891,-13.3498148582613));
#82917=CARTESIAN_POINT('Ctrl Pts',(18.0623711506552,-20.9596395277255,-13.3500310793731));
#82918=CARTESIAN_POINT('Ctrl Pts',(18.0551094862089,-20.957196590331,-13.3504955064512));
#82919=CARTESIAN_POINT('Ctrl Pts',(18.0512405574551,-20.9558825411071,-13.3507438590022));
#82920=CARTESIAN_POINT('Ctrl Pts',(18.0406289262692,-20.9522440904301,-13.3514274927815));
#82921=CARTESIAN_POINT('Ctrl Pts',(18.0338942003764,-20.949896827462,-13.3518640934334));
#82922=CARTESIAN_POINT('Ctrl Pts',(17.9984774555781,-20.937351918409,-13.3541740180201));
#82923=CARTESIAN_POINT('Ctrl Pts',(17.9700075772509,-20.9265710947681,-13.3560790445638));
#82924=CARTESIAN_POINT('Ctrl Pts',(17.7914208839187,-20.8545045692563,-13.3682924779572));
#82925=CARTESIAN_POINT('Ctrl Pts',(17.648533283028,-20.776757592915,-13.3792084718668));
#82926=CARTESIAN_POINT('Ctrl Pts',(17.4180928158084,-20.6146437362195,-13.3976307292246));
#82927=CARTESIAN_POINT('Ctrl Pts',(17.3262603531878,-20.5376460354167,-13.4052583400663));
#82928=CARTESIAN_POINT('Ctrl Pts',(17.2302711961142,-20.4422132351479,-13.4135235262956));
#82929=CARTESIAN_POINT('Ctrl Pts',(17.2192537705425,-20.4310130773836,-13.4144773329668));
#82930=CARTESIAN_POINT('Ctrl Pts',(17.2027731928931,-20.4138818164368,-13.4159122608872));
#82931=CARTESIAN_POINT('Ctrl Pts',(17.1972177502792,-20.4080406243576,-13.4163973987769));
#82932=CARTESIAN_POINT('Ctrl Pts',(17.1873222616745,-20.3975164254442,-13.4172641882906));
#82933=CARTESIAN_POINT('Ctrl Pts',(17.1829698046474,-20.3928452716892,-13.4176463725963));
#82934=CARTESIAN_POINT('Ctrl Pts',(17.17377904543,-20.3828916397041,-13.4184554318016));
#82935=CARTESIAN_POINT('Ctrl Pts',(17.168946279822,-20.3776041408986,-13.4188820679075));
#82936=CARTESIAN_POINT('Ctrl Pts',(17.1591628939954,-20.3667904910308,-13.4197482784963));
#82937=CARTESIAN_POINT('Ctrl Pts',(17.1542142980577,-20.3612626377019,-13.4201877647381));
#82938=CARTESIAN_POINT('Ctrl Pts',(17.1324256429663,-20.3366645202445,-13.4221289594741));
#82939=CARTESIAN_POINT('Ctrl Pts',(17.1159006368997,-20.3173171016113,-13.4236175617699));
#82940=CARTESIAN_POINT('Ctrl Pts',(17.0457285969941,-20.2320958290432,-13.4300186821377));
#82941=CARTESIAN_POINT('Ctrl Pts',(16.9957224725482,-20.1633212222884,-13.4347859059221));
#82942=CARTESIAN_POINT('Ctrl Pts',(16.9128101395665,-20.0335375559321,-13.4432735523562));
#82943=CARTESIAN_POINT('Ctrl Pts',(16.8785074225223,-19.9735692052281,-13.4470186833148));
#82944=CARTESIAN_POINT('Ctrl Pts',(16.8085769131631,-19.8361307746912,-13.4553932932223));
#82945=CARTESIAN_POINT('Ctrl Pts',(16.7745951536274,-19.7580132150682,-13.460014549721));
#82946=CARTESIAN_POINT('Ctrl Pts',(16.7454194853472,-19.6781105540779,-13.4647888353055));
#82947=CARTESIAN_POINT('',(16.6170008459317,-18.9538925311169,-12.4890563034236));
#82948=CARTESIAN_POINT('Ctrl Pts',(16.7454194499637,-19.6781104571739,-13.2445592876386));
#82949=CARTESIAN_POINT('Ctrl Pts',(16.7717392418346,-19.7501918129489,-13.2399327110257));
#82950=CARTESIAN_POINT('Ctrl Pts',(16.8019456368363,-19.820740464874,-13.2353061344128));
#82951=CARTESIAN_POINT('Ctrl Pts',(16.8358258581282,-19.8893494157086,-13.2306795577999));
#82952=CARTESIAN_POINT('Ctrl Pts',(16.8465556082421,-19.911077635595,-13.229214336823));
#82953=CARTESIAN_POINT('Ctrl Pts',(16.8576534978601,-19.9326115175269,-13.2277491158461));
#82954=CARTESIAN_POINT('Ctrl Pts',(16.8691118619909,-19.9539387370059,-13.2262838948692));
#82955=CARTESIAN_POINT('Ctrl Pts',(16.9034286623953,-20.017811897754,-13.2218956859383));
#82956=CARTESIAN_POINT('Ctrl Pts',(16.9410977666971,-20.0800446523181,-13.2175074770074));
#82957=CARTESIAN_POINT('Ctrl Pts',(16.9819381659419,-20.1402627359456,-13.2131192680765));
#82958=CARTESIAN_POINT('Ctrl Pts',(17.0227179512628,-20.2003914459526,-13.2087375719752));
#82959=CARTESIAN_POINT('Ctrl Pts',(17.0666594195118,-20.2585110248676,-13.2043558758739));
#82960=CARTESIAN_POINT('Ctrl Pts',(17.1135357879723,-20.3142719029391,-13.1999741797727));
#82961=CARTESIAN_POINT('Ctrl Pts',(17.1603570729693,-20.3699672575413,-13.195597632513));
#82962=CARTESIAN_POINT('Ctrl Pts',(17.2101060983655,-20.4233090498181,-13.1912210852534));
#82963=CARTESIAN_POINT('Ctrl Pts',(17.2625139124404,-20.4739782173601,-13.1868445379937));
#82964=CARTESIAN_POINT('Ctrl Pts',(17.3148884902414,-20.5246152512525,-13.1824707662767));
#82965=CARTESIAN_POINT('Ctrl Pts',(17.3699181652074,-20.5725826889237,-13.1780969945598));
#82966=CARTESIAN_POINT('Ctrl Pts',(17.427295955156,-20.6175970518671,-13.1737232228428));
#82967=CARTESIAN_POINT('Ctrl Pts',(17.4846562848506,-20.6625977167887,-13.1693507820792));
#82968=CARTESIAN_POINT('Ctrl Pts',(17.5443629316538,-20.7046467934755,-13.1649783413157));
#82969=CARTESIAN_POINT('Ctrl Pts',(17.6060758346845,-20.743501068182,-13.1606059005521));
#82970=CARTESIAN_POINT('Ctrl Pts',(17.667790315721,-20.7823563363967,-13.1562333479848));
#82971=CARTESIAN_POINT('Ctrl Pts',(17.7315107455617,-20.8180163851248,-13.1518607954174));
#82972=CARTESIAN_POINT('Ctrl Pts',(17.7968695201153,-20.8502822402559,-13.1474882428501));
#82973=CARTESIAN_POINT('Ctrl Pts',(17.8622961264704,-20.8825815821085,-13.1431111522827));
#82974=CARTESIAN_POINT('Ctrl Pts',(17.9293640389074,-20.9114794832211,-13.1387340617154));
#82975=CARTESIAN_POINT('Ctrl Pts',(17.9976833250409,-20.9368241116475,-13.134356971148));
#82976=CARTESIAN_POINT('Ctrl Pts',(18.0660399228722,-20.9621825817161,-13.1299774900891));
#82977=CARTESIAN_POINT('Ctrl Pts',(18.135648794438,-20.9839837711618,-13.1255980090301));
#82978=CARTESIAN_POINT('Ctrl Pts',(18.2061050046745,-21.0021258190439,-13.1212185279712));
#82979=CARTESIAN_POINT('Ctrl Pts',(18.2766860980708,-21.0203000235841,-13.1168312843115));
#82980=CARTESIAN_POINT('Ctrl Pts',(18.3481170562253,-21.0348020386144,-13.1124440406517));
#82981=CARTESIAN_POINT('Ctrl Pts',(18.4199835016935,-21.0455812950042,-13.108056796992));
#82982=CARTESIAN_POINT('Ctrl Pts',(18.4688457595767,-21.0529101506624,-13.1050738940573));
#82983=CARTESIAN_POINT('Ctrl Pts',(18.517909182164,-21.0585191746184,-13.1020909911225));
#82984=CARTESIAN_POINT('Ctrl Pts',(18.5670433388759,-21.0624062341896,-13.0991080881877));
#82985=CARTESIAN_POINT('Ctrl Pts',(18.6393255921073,-21.0681245662635,-13.0947198792568));
#82986=CARTESIAN_POINT('Ctrl Pts',(18.7120430618562,-21.0701362205188,-13.0903316703259));
#82987=CARTESIAN_POINT('Ctrl Pts',(18.7847830739802,-21.0683908144285,-13.085943461395));
#82988=CARTESIAN_POINT('Ctrl Pts',(18.8574151278658,-21.0666479988102,-13.0815617652938));
#82989=CARTESIAN_POINT('Ctrl Pts',(18.9300691794577,-21.0611592036426,-13.0771800691925));
#82990=CARTESIAN_POINT('Ctrl Pts',(19.0023285427326,-21.0519259018249,-13.0727983730912));
#82991=CARTESIAN_POINT('Ctrl Pts',(19.074502995505,-21.0427034498716,-13.0684218258316));
#82992=CARTESIAN_POINT('Ctrl Pts',(19.14628320517,-21.0297452929198,-13.064045278572));
#82993=CARTESIAN_POINT('Ctrl Pts',(19.2172553122691,-21.0131048743729,-13.0596687313123));
#82994=CARTESIAN_POINT('Ctrl Pts',(19.2881824098894,-20.9964750089376,-13.0552949595954));
#82995=CARTESIAN_POINT('Ctrl Pts',(19.358301953298,-20.9761676251632,-13.0509211878784));
#82996=CARTESIAN_POINT('Ctrl Pts',(19.4272094182993,-20.9522874049449,-13.0465474161614));
#82997=CARTESIAN_POINT('Ctrl Pts',(19.4960959145276,-20.9284144515578,-13.0421749753979));
#82998=CARTESIAN_POINT('Ctrl Pts',(19.563770609099,-20.9009709780648,-13.0378025346343));
#82999=CARTESIAN_POINT('Ctrl Pts',(19.6298449292376,-20.8701112748637,-13.0334300938708));
#83000=CARTESIAN_POINT('Ctrl Pts',(19.6959209389039,-20.8392507825766,-13.0290575413034));
#83001=CARTESIAN_POINT('Ctrl Pts',(19.7603960566783,-20.8049740930876,-13.0246849887361));
#83002=CARTESIAN_POINT('Ctrl Pts',(19.8229039996999,-20.7674826023506,-13.0203124361687));
#83003=CARTESIAN_POINT('Ctrl Pts',(19.8854768158225,-20.7299522015303,-13.0159353456014));
#83004=CARTESIAN_POINT('Ctrl Pts',(19.9460779664247,-20.6892005866783,-13.0115582550341));
#83005=CARTESIAN_POINT('Ctrl Pts',(20.0043687218632,-20.6454734454699,-13.0071811644668));
#83006=CARTESIAN_POINT('Ctrl Pts',(20.0626913120466,-20.6017224232467,-13.0028016834078));
#83007=CARTESIAN_POINT('Ctrl Pts',(20.1187006241993,-20.5549929484574,-12.9984222023489));
#83008=CARTESIAN_POINT('Ctrl Pts',(20.1720918257202,-20.505570372013,-12.9940427212899));
#83009=CARTESIAN_POINT('Ctrl Pts',(20.2255776627874,-20.4560601943837,-12.9896554776302));
#83010=CARTESIAN_POINT('Ctrl Pts',(20.276435785288,-20.4038477284535,-12.9852682339705));
#83011=CARTESIAN_POINT('Ctrl Pts',(20.3243993779345,-20.3492540279655,-12.9808809903108));
#83012=CARTESIAN_POINT('Ctrl Pts',(20.3570099991733,-20.3121355722701,-12.977898087376));
#83013=CARTESIAN_POINT('Ctrl Pts',(20.3882834007586,-20.2739170566123,-12.9749151844411));
#83014=CARTESIAN_POINT('Ctrl Pts',(20.4181471898432,-20.2347069980878,-12.9719322815063));
#83015=CARTESIAN_POINT('Ctrl Pts',(20.4620804149045,-20.1770242867296,-12.9675440725754));
#83016=CARTESIAN_POINT('Ctrl Pts',(20.5031324849612,-20.1169692727542,-12.9631558636445));
#83017=CARTESIAN_POINT('Ctrl Pts',(20.541037663595,-20.0548616787019,-12.9587676547136));
#83018=CARTESIAN_POINT('Ctrl Pts',(20.578886584659,-19.9928462626168,-12.9543859586124));
#83019=CARTESIAN_POINT('Ctrl Pts',(20.6135976366773,-19.9287847222599,-12.9500042625111));
#83020=CARTESIAN_POINT('Ctrl Pts',(20.6449465138838,-19.8630282218874,-12.9456225664098));
#83021=CARTESIAN_POINT('Ctrl Pts',(20.6762585536647,-19.7973489906359,-12.9412460191502));
#83022=CARTESIAN_POINT('Ctrl Pts',(20.7042160604134,-19.7299791891849,-12.9368694718905));
#83023=CARTESIAN_POINT('Ctrl Pts',(20.728639957299,-19.661295735745,-12.9324929246309));
#83024=CARTESIAN_POINT('Ctrl Pts',(20.7530483649043,-19.5926558403532,-12.9281191529139));
#83025=CARTESIAN_POINT('Ctrl Pts',(20.7739274477879,-19.5227043993277,-12.9237453811969));
#83026=CARTESIAN_POINT('Ctrl Pts',(20.7911462655829,-19.4518382158243,-12.91937160948));
#83027=CARTESIAN_POINT('Ctrl Pts',(20.8083598436337,-19.3809935971386,-12.9149991687164));
#83028=CARTESIAN_POINT('Ctrl Pts',(20.8219152540694,-19.3092352570616,-12.9106267279528));
#83029=CARTESIAN_POINT('Ctrl Pts',(20.8317319036236,-19.2369734382707,-12.9062542871893));
#83030=CARTESIAN_POINT('Ctrl Pts',(20.8415488041906,-19.1647097717371,-12.9018817346219));
#83031=CARTESIAN_POINT('Ctrl Pts',(20.847626691118,-19.0919430791858,-12.8975091820546));
#83032=CARTESIAN_POINT('Ctrl Pts',(20.8499366445659,-19.0190903583475,-12.8931366294872));
#83033=CARTESIAN_POINT('Ctrl Pts',(20.8522489953706,-18.9461620282076,-12.8887595389199));
#83034=CARTESIAN_POINT('Ctrl Pts',(20.8507855897922,-18.8731479746872,-12.8843824483526));
#83035=CARTESIAN_POINT('Ctrl Pts',(20.8455696643532,-18.8004660018902,-12.8800053577853));
#83036=CARTESIAN_POINT('Ctrl Pts',(20.8403508903038,-18.7277443347703,-12.8756258767263));
#83037=CARTESIAN_POINT('Ctrl Pts',(20.8313755754733,-18.6553555885068,-12.8712463956674));
#83038=CARTESIAN_POINT('Ctrl Pts',(20.8187186547149,-18.5837105341125,-12.8668669146084));
#83039=CARTESIAN_POINT('Ctrl Pts',(20.8060392996494,-18.5119384893402,-12.8624796709487));
#83040=CARTESIAN_POINT('Ctrl Pts',(20.789665415713,-18.4409132392693,-12.858092427289));
#83041=CARTESIAN_POINT('Ctrl Pts',(20.769722536241,-18.371032913634,-12.8537051836293));
#83042=CARTESIAN_POINT('Ctrl Pts',(20.7561632998913,-18.3235210258541,-12.8507222806944));
#83043=CARTESIAN_POINT('Ctrl Pts',(20.7409552755656,-18.27653808659,-12.8477393777596));
#83044=CARTESIAN_POINT('Ctrl Pts',(20.7241505240927,-18.2302037050152,-12.8447564748248));
#83045=CARTESIAN_POINT('Ctrl Pts',(20.6994287137936,-18.1620402577033,-12.8403682658939));
#83046=CARTESIAN_POINT('Ctrl Pts',(20.6711526578599,-18.0950153233851,-12.835980056963));
#83047=CARTESIAN_POINT('Ctrl Pts',(20.6394473542677,-18.0295254040819,-12.8315918480321));
#83048=CARTESIAN_POINT('Ctrl Pts',(20.6077891066029,-17.9641326826773,-12.8272101519309));
#83049=CARTESIAN_POINT('Ctrl Pts',(20.5727119232316,-17.9002708843009,-12.8228284558296));
#83050=CARTESIAN_POINT('Ctrl Pts',(20.5343896652636,-17.8383186931567,-12.8184467597283));
#83051=CARTESIAN_POINT('Ctrl Pts',(20.4961124389984,-17.7764393007675,-12.8140702124687));
#83052=CARTESIAN_POINT('Ctrl Pts',(20.4545979656273,-17.7164654662072,-12.8096936652091));
#83053=CARTESIAN_POINT('Ctrl Pts',(20.410066242825,-17.6587517834296,-12.8053171179494));
#83054=CARTESIAN_POINT('Ctrl Pts',(20.365562761394,-17.6010747018308,-12.8009433462325));
#83055=CARTESIAN_POINT('Ctrl Pts',(20.318046121109,-17.5456553090191,-12.7965695745155));
#83056=CARTESIAN_POINT('Ctrl Pts',(20.2677790950911,-17.4928184871437,-12.7921958027985));
#83057=CARTESIAN_POINT('Ctrl Pts',(20.217527365498,-17.4399977436906,-12.787823362035));
#83058=CARTESIAN_POINT('Ctrl Pts',(20.1645272440669,-17.3897583602253,-12.7834509212714));
#83059=CARTESIAN_POINT('Ctrl Pts',(20.1090800563607,-17.342390159511,-12.7790784805079));
#83060=CARTESIAN_POINT('Ctrl Pts',(20.0536314508638,-17.2950207475865,-12.7747059279405));
#83061=CARTESIAN_POINT('Ctrl Pts',(19.9957360229245,-17.2505229759785,-12.7703333753732));
#83062=CARTESIAN_POINT('Ctrl Pts',(19.9357287478822,-17.2091468746583,-12.7659608228059));
#83063=CARTESIAN_POINT('Ctrl Pts',(19.8756591950264,-17.1677278316594,-12.7615837322385));
#83064=CARTESIAN_POINT('Ctrl Pts',(19.8134738170564,-17.1294372018124,-12.7572066416712));
#83065=CARTESIAN_POINT('Ctrl Pts',(19.7495364985935,-17.0944815963161,-12.7528295511039));
#83066=CARTESIAN_POINT('Ctrl Pts',(19.6855642615879,-17.0595069002662,-12.7484500700449));
#83067=CARTESIAN_POINT('Ctrl Pts',(19.6198386140604,-17.027871064273,-12.744070588986));
#83068=CARTESIAN_POINT('Ctrl Pts',(19.5527455102415,-16.999733422542,-12.7396911079271));
#83069=CARTESIAN_POINT('Ctrl Pts',(19.4855334843464,-16.9715459070299,-12.7353038642674));
#83070=CARTESIAN_POINT('Ctrl Pts',(19.4169496162068,-16.9468691314342,-12.7309166206076));
#83071=CARTESIAN_POINT('Ctrl Pts',(19.3473966187373,-16.9258130421598,-12.7265293769479));
#83072=CARTESIAN_POINT('Ctrl Pts',(19.3001072825687,-16.9114969304131,-12.7235464740131));
#83073=CARTESIAN_POINT('Ctrl Pts',(19.2523702507342,-16.8988534982272,-12.7205635710783));
#83074=CARTESIAN_POINT('Ctrl Pts',(19.2043142751595,-16.8879037128609,-12.7175806681434));
#83075=CARTESIAN_POINT('Ctrl Pts',(19.1336181560408,-16.8717952618032,-12.7131924592126));
#83076=CARTESIAN_POINT('Ctrl Pts',(19.061955500426,-16.8592916243426,-12.7088042502817));
#83077=CARTESIAN_POINT('Ctrl Pts',(18.9897273628005,-16.8505023159863,-12.7044160413508));
#83078=CARTESIAN_POINT('Ctrl Pts',(18.917606423707,-16.8417260524208,-12.7000343452495));
#83079=CARTESIAN_POINT('Ctrl Pts',(18.8449221435538,-16.8366532323251,-12.6956526491482));
#83080=CARTESIAN_POINT('Ctrl Pts',(18.7720870435493,-16.8353426405973,-12.691270953047));
#83081=CARTESIAN_POINT('Ctrl Pts',(18.6993375305838,-16.8340335889191,-12.6868944057873));
#83082=CARTESIAN_POINT('Ctrl Pts',(18.6264380297321,-16.8364779920626,-12.6825178585277));
#83083=CARTESIAN_POINT('Ctrl Pts',(18.5538057789625,-16.8426828017805,-12.6781413112681));
#83084=CARTESIAN_POINT('Ctrl Pts',(18.4812195905107,-16.8488836764982,-12.6737675395511));
#83085=CARTESIAN_POINT('Ctrl Pts',(18.4089007953032,-16.8588401850895,-12.6693937678341));
#83086=CARTESIAN_POINT('Ctrl Pts',(18.3372648019203,-16.8725072294897,-12.6650199961172));
#83087=CARTESIAN_POINT('Ctrl Pts',(18.2656506076109,-16.8861701149623,-12.6606475553536));
#83088=CARTESIAN_POINT('Ctrl Pts',(18.1947192761675,-16.9035412042303,-12.6562751145901));
#83089=CARTESIAN_POINT('Ctrl Pts',(18.1248776044808,-16.9245240057458,-12.6519026738265));
#83090=CARTESIAN_POINT('Ctrl Pts',(18.0550341469347,-16.9455073437939,-12.6475301212592));
#83091=CARTESIAN_POINT('Ctrl Pts',(17.9862808658674,-16.9701024367363,-12.6431575686918));
#83092=CARTESIAN_POINT('Ctrl Pts',(17.9190093127146,-16.998162959805,-12.6387850161245));
#83093=CARTESIAN_POINT('Ctrl Pts',(17.8516679426066,-17.0262526051429,-12.6344079255571));
#83094=CARTESIAN_POINT('Ctrl Pts',(17.7858118168726,-17.0578146752693,-12.6300308349898));
#83095=CARTESIAN_POINT('Ctrl Pts',(17.7218116266778,-17.0926550355269,-12.6256537444225));
#83096=CARTESIAN_POINT('Ctrl Pts',(17.6577764836039,-17.1275144233984,-12.6212742633635));
#83097=CARTESIAN_POINT('Ctrl Pts',(17.5955997055921,-17.1656554136578,-12.6168947823046));
#83098=CARTESIAN_POINT('Ctrl Pts',(17.5356241771988,-17.2068397244592,-12.6125153012457));
#83099=CARTESIAN_POINT('Ctrl Pts',(17.475542342584,-17.2480970341751,-12.6081280575859));
#83100=CARTESIAN_POINT('Ctrl Pts',(17.4176699324644,-17.2924081430501,-12.6037408139262));
#83101=CARTESIAN_POINT('Ctrl Pts',(17.3623173752297,-17.3394939451577,-12.5993535702665));
#83102=CARTESIAN_POINT('Ctrl Pts',(17.3246829700697,-17.3715077534138,-12.5963706673317));
#83103=CARTESIAN_POINT('Ctrl Pts',(17.2882126945402,-17.404803392597,-12.5933877643969));
#83104=CARTESIAN_POINT('Ctrl Pts',(17.2529938697634,-17.4392839518926,-12.590404861462));
#83105=CARTESIAN_POINT('Ctrl Pts',(17.2019441492123,-17.4892635559153,-12.5860811407752));
#83106=CARTESIAN_POINT('Ctrl Pts',(17.1533139178898,-17.5419415318573,-12.5817574200883));
#83107=CARTESIAN_POINT('Ctrl Pts',(17.1074080252024,-17.5970507214202,-12.5774336994015));
#83108=CARTESIAN_POINT('Ctrl Pts',(17.061563088785,-17.652086734089,-12.5731157199795));
#83109=CARTESIAN_POINT('Ctrl Pts',(17.0184356374498,-17.7095471849219,-12.5687977405574));
#83110=CARTESIAN_POINT('Ctrl Pts',(16.9782947055966,-17.7691272599286,-12.5644797611354));
#83111=CARTESIAN_POINT('Ctrl Pts',(16.9381929308678,-17.8286492150987,-12.5601659938641));
#83112=CARTESIAN_POINT('Ctrl Pts',(16.9010721765566,-17.8902862851977,-12.5558522265929));
#83113=CARTESIAN_POINT('Ctrl Pts',(16.8671608676011,-17.9537011200325,-12.5515384593216));
#83114=CARTESIAN_POINT('Ctrl Pts',(16.8332706976895,-18.0170764244272,-12.5472273810918));
#83115=CARTESIAN_POINT('Ctrl Pts',(16.8025862384805,-18.0822268576,-12.542916302862));
#83116=CARTESIAN_POINT('Ctrl Pts',(16.7752912625976,-18.1487882707382,-12.5386052246321));
#83117=CARTESIAN_POINT('Ctrl Pts',(16.7479923079761,-18.2153593864121,-12.5342935179843));
#83118=CARTESIAN_POINT('Ctrl Pts',(16.7240840285399,-18.2833414390349,-12.5299818113365));
#83119=CARTESIAN_POINT('Ctrl Pts',(16.7037024934055,-18.3523492393766,-12.5256701046887));
#83120=CARTESIAN_POINT('Ctrl Pts',(16.6833204782339,-18.4213586650285,-12.5213582964892));
#83121=CARTESIAN_POINT('Ctrl Pts',(16.6664655033666,-18.4913934058167,-12.5170464882897));
#83122=CARTESIAN_POINT('Ctrl Pts',(16.6532233605848,-18.5620543924288,-12.5127346800901));
#83123=CARTESIAN_POINT('Ctrl Pts',(16.639966456221,-18.6327941478605,-12.5084180653339));
#83124=CARTESIAN_POINT('Ctrl Pts',(16.6303305065811,-18.7041610510436,-12.5041014505776));
#83125=CARTESIAN_POINT('Ctrl Pts',(16.6243497245845,-18.7757481477001,-12.4997848358213));
#83126=CARTESIAN_POINT('Ctrl Pts',(16.6193948377084,-18.8350557710035,-12.4962086583554));
#83127=CARTESIAN_POINT('Ctrl Pts',(16.6169477636251,-18.8945142745606,-12.4926324808895));
#83128=CARTESIAN_POINT('Ctrl Pts',(16.6170008459317,-18.9538925311169,-12.4890563034236));
#83129=CARTESIAN_POINT('Ctrl Pts',(16.6163526597653,-18.9538935158516,-12.4890562790225));
#83130=CARTESIAN_POINT('Ctrl Pts',(16.6150299521963,-19.0968822256806,-12.4804472042752));
#83131=CARTESIAN_POINT('Ctrl Pts',(16.6379358826496,-19.3437931578393,-12.4655558028313));
#83132=CARTESIAN_POINT('Ctrl Pts',(16.7071054598744,-19.5811888020602,-12.4506644013873));
#83133=CARTESIAN_POINT('Ctrl Pts',(16.7437496527793,-19.6787359237804,-12.4443820746906));
#83134=CARTESIAN_POINT('Origin',(18.734,-18.952,0.));
#83135=CARTESIAN_POINT('',(16.7454194494007,-19.678110455632,-11.6425492951846));
#83136=CARTESIAN_POINT('',(16.7454194500115,-19.678110457305,-11.8674650116542));
#83137=CARTESIAN_POINT('',(16.7454194499637,-19.6781104571739,0.));
#83138=CARTESIAN_POINT('',(16.6170006007775,-18.9504051045321,-11.9120634828057));
#83139=CARTESIAN_POINT('Ctrl Pts',(16.7454194500115,-19.678110457305,-11.8674650116542));
#83140=CARTESIAN_POINT('Ctrl Pts',(16.7321284699056,-19.6417107824854,-11.8699797021076));
#83141=CARTESIAN_POINT('Ctrl Pts',(16.7198387408441,-19.6049512409371,-11.8724726322167));
#83142=CARTESIAN_POINT('Ctrl Pts',(16.705693847586,-19.5584326133417,-11.8755657202205));
#83143=CARTESIAN_POINT('Ctrl Pts',(16.7028892951475,-19.548972086202,-11.8761916170213));
#83144=CARTESIAN_POINT('Ctrl Pts',(16.684621334253,-19.4857299258936,-11.8803545370693));
#83145=CARTESIAN_POINT('Ctrl Pts',(16.6712284886434,-19.4313695483551,-11.8838303862752));
#83146=CARTESIAN_POINT('Ctrl Pts',(16.6575927142468,-19.3647547060886,-11.8879694847778));
#83147=CARTESIAN_POINT('Ctrl Pts',(16.655281149068,-19.3529508846168,-11.8886984191902));
#83148=CARTESIAN_POINT('Ctrl Pts',(16.6516247940173,-19.3333978798055,-11.889898626918));
#83149=CARTESIAN_POINT('Ctrl Pts',(16.6502223868832,-19.3256598759411,-11.8903717274574));
#83150=CARTESIAN_POINT('Ctrl Pts',(16.6477625561846,-19.3116426982719,-11.8912254000915));
#83151=CARTESIAN_POINT('Ctrl Pts',(16.6466902882239,-19.3053662560213,-11.8916064401833));
#83152=CARTESIAN_POINT('Ctrl Pts',(16.6446635443308,-19.2931716702623,-11.8923444618685));
#83153=CARTESIAN_POINT('Ctrl Pts',(16.6437058571057,-19.2872541288255,-11.8927015420183));
#83154=CARTESIAN_POINT('Ctrl Pts',(16.6416603283115,-19.2742652384781,-11.8934830566531));
#83155=CARTESIAN_POINT('Ctrl Pts',(16.6405831698579,-19.2671922632905,-11.8939071501069));
#83156=CARTESIAN_POINT('Ctrl Pts',(16.6380228005234,-19.2497877047711,-11.8949471799295));
#83157=CARTESIAN_POINT('Ctrl Pts',(16.6365800904223,-19.2394502853674,-11.8955618403836));
#83158=CARTESIAN_POINT('Ctrl Pts',(16.6230153964929,-19.136710708443,-11.9016413870128));
#83159=CARTESIAN_POINT('Ctrl Pts',(16.6169303820547,-19.043610582272,-11.9069087499733));
#83160=CARTESIAN_POINT('Ctrl Pts',(16.6170006007775,-18.9504051045321,-11.9120634828057));
#83161=CARTESIAN_POINT('Ctrl Pts',(16.6170005988957,-18.9504076043165,-11.912063344555));
#83162=CARTESIAN_POINT('Ctrl Pts',(16.6171142130127,-18.7993641041209,-11.9204168148733));
#83163=CARTESIAN_POINT('Ctrl Pts',(16.6333918366525,-18.6487693419506,-11.9284162966799));
#83164=CARTESIAN_POINT('Ctrl Pts',(16.6785865590018,-18.4414036071667,-11.9402353573198));
#83165=CARTESIAN_POINT('Ctrl Pts',(16.6942013609097,-18.3822165259633,-11.9437094928887));
#83166=CARTESIAN_POINT('Ctrl Pts',(16.7161304297539,-18.3116460075593,-11.9480644897593));
#83167=CARTESIAN_POINT('Ctrl Pts',(16.7200147926183,-18.2995320660581,-11.9488197826088));
#83168=CARTESIAN_POINT('Ctrl Pts',(16.725627212657,-18.2825566830156,-11.9498900318538));
#83169=CARTESIAN_POINT('Ctrl Pts',(16.7272643113937,-18.2776651555869,-11.9501998191164));
#83170=CARTESIAN_POINT('Ctrl Pts',(16.7300928755629,-18.2693151405452,-11.9507310945633));
#83171=CARTESIAN_POINT('Ctrl Pts',(16.7312754716076,-18.26585362795,-11.9509520600016));
#83172=CARTESIAN_POINT('Ctrl Pts',(16.7335672004791,-18.259202034274,-11.9513780874896));
#83173=CARTESIAN_POINT('Ctrl Pts',(16.7346750010501,-18.2560115267365,-11.951583065312));
#83174=CARTESIAN_POINT('Ctrl Pts',(16.7376455275145,-18.2475219161551,-11.9521301409547));
#83175=CARTESIAN_POINT('Ctrl Pts',(16.7395217014979,-18.2422275959306,-11.9524730262259));
#83176=CARTESIAN_POINT('Ctrl Pts',(16.7463383467246,-18.2232323576625,-11.9537092606304));
#83177=CARTESIAN_POINT('Ctrl Pts',(16.7513989781569,-18.2095754005923,-11.9546093395308));
#83178=CARTESIAN_POINT('Ctrl Pts',(16.8132024685467,-18.0479276115216,-11.9653881411684));
#83179=CARTESIAN_POINT('Ctrl Pts',(16.8862469759508,-17.9067188523124,-11.976016176932));
#83180=CARTESIAN_POINT('Ctrl Pts',(17.0125880598064,-17.7178369517081,-11.9909701619109));
#83181=CARTESIAN_POINT('Ctrl Pts',(17.0535836430284,-17.6625739634773,-11.9954558897231));
#83182=CARTESIAN_POINT('Ctrl Pts',(17.1293346621576,-17.5702237030643,-12.0031050472166));
#83183=CARTESIAN_POINT('Ctrl Pts',(17.1628683974291,-17.532210326528,-12.0063038104558));
#83184=CARTESIAN_POINT('Ctrl Pts',(17.2125182539898,-17.4798438011907,-12.0107814371134));
#83185=CARTESIAN_POINT('Ctrl Pts',(17.2275370702007,-17.4644785476137,-12.0121046145792));
#83186=CARTESIAN_POINT('Ctrl Pts',(17.2544659617231,-17.4377547334978,-12.0144231779045));
#83187=CARTESIAN_POINT('Ctrl Pts',(17.2662792517708,-17.4263016265491,-12.0154226706571));
#83188=CARTESIAN_POINT('Ctrl Pts',(17.2841042396734,-17.4094187687792,-12.0169051143085));
#83189=CARTESIAN_POINT('Ctrl Pts',(17.2900153133673,-17.4038841134003,-12.0173925967246));
#83190=CARTESIAN_POINT('Ctrl Pts',(17.3006606305797,-17.3940307087213,-12.0182632244455));
#83191=CARTESIAN_POINT('Ctrl Pts',(17.3053829764859,-17.3896993048638,-12.018646908923));
#83192=CARTESIAN_POINT('Ctrl Pts',(17.3146944928213,-17.3812361708287,-12.0193985407608));
#83193=CARTESIAN_POINT('Ctrl Pts',(17.3192822152422,-17.3771029492464,-12.0197665493077));
#83194=CARTESIAN_POINT('Ctrl Pts',(17.3318231016589,-17.3659034935425,-12.0207662977765));
#83195=CARTESIAN_POINT('Ctrl Pts',(17.3398116206925,-17.3588769817433,-12.0213963690959));
#83196=CARTESIAN_POINT('Ctrl Pts',(17.3705138519407,-17.3322798321615,-12.0237926510791));
#83197=CARTESIAN_POINT('Ctrl Pts',(17.3935900721898,-17.3131317148734,-12.0255414533878));
#83198=CARTESIAN_POINT('Ctrl Pts',(17.4221564830299,-17.2904351184303,-12.0276474036579));
#83199=CARTESIAN_POINT('Ctrl Pts',(17.4272654717086,-17.2864141743747,-12.0280218100182));
#83200=CARTESIAN_POINT('Ctrl Pts',(17.5660775382317,-17.178196287701,-12.0381351746127));
#83201=CARTESIAN_POINT('Ctrl Pts',(17.7117917382368,-17.0904101355843,-12.0472020282944));
#83202=CARTESIAN_POINT('Ctrl Pts',(17.9387511016617,-16.9884432036371,-12.0607697065465));
#83203=CARTESIAN_POINT('Ctrl Pts',(18.0128412415804,-16.9600401139217,-12.0651327156219));
#83204=CARTESIAN_POINT('Ctrl Pts',(18.1224372702966,-16.9249426107655,-12.0717169269656));
#83205=CARTESIAN_POINT('Ctrl Pts',(18.1568007474809,-16.9148914334043,-12.0737996388527));
#83206=CARTESIAN_POINT('Ctrl Pts',(18.1986034450125,-16.9038068780349,-12.0763734115849));
#83207=CARTESIAN_POINT('Ctrl Pts',(18.2058166669621,-16.901934903738,-12.0768189588341));
#83208=CARTESIAN_POINT('Ctrl Pts',(18.2170679587025,-16.899078291979,-12.0775163727656));
#83209=CARTESIAN_POINT('Ctrl Pts',(18.2210993807744,-16.8980673748393,-12.0777667485368));
#83210=CARTESIAN_POINT('Ctrl Pts',(18.2285953757885,-16.8962111286051,-12.0782332440898));
#83211=CARTESIAN_POINT('Ctrl Pts',(18.2320591170933,-16.8953626796677,-12.0784491813962));
#83212=CARTESIAN_POINT('Ctrl Pts',(18.2399127524657,-16.8934599410253,-12.0789396480693));
#83213=CARTESIAN_POINT('Ctrl Pts',(18.2443038634695,-16.8924109449763,-12.0792144763959));
#83214=CARTESIAN_POINT('Ctrl Pts',(18.2556574693868,-16.8897370341274,-12.0799265564264));
#83215=CARTESIAN_POINT('Ctrl Pts',(18.2626248351889,-16.8881333454716,-12.0803649808801));
#83216=CARTESIAN_POINT('Ctrl Pts',(18.3056159411292,-16.87846706869,-12.0830785254479));
#83217=CARTESIAN_POINT('Ctrl Pts',(18.3418350182682,-16.8713131024546,-12.0854004639583));
#83218=CARTESIAN_POINT('Ctrl Pts',(18.546300494839,-16.8364551336416,-12.0986400980833));
#83219=CARTESIAN_POINT('Ctrl Pts',(18.7172256339539,-16.8282102320616,-12.1101449892438));
#83220=CARTESIAN_POINT('Ctrl Pts',(18.9821998790576,-16.8474476453823,-12.1274081236477));
#83221=CARTESIAN_POINT('Ctrl Pts',(19.0765437542806,-16.8607296223075,-12.1334532439658));
#83222=CARTESIAN_POINT('Ctrl Pts',(19.1905921974845,-16.8847145815008,-12.1406117801762));
#83223=CARTESIAN_POINT('Ctrl Pts',(19.2114320464133,-16.8894277879518,-12.1419139966346));
#83224=CARTESIAN_POINT('Ctrl Pts',(19.2409498845181,-16.8965750054515,-12.1437507242227));
#83225=CARTESIAN_POINT('Ctrl Pts',(19.2496886666514,-16.8987500647432,-12.1442935200281));
#83226=CARTESIAN_POINT('Ctrl Pts',(19.2647355391844,-16.9025973139173,-12.145226534528));
#83227=CARTESIAN_POINT('Ctrl Pts',(19.2710502136786,-16.9042430193638,-12.1456176025372));
#83228=CARTESIAN_POINT('Ctrl Pts',(19.2831230418729,-16.9074490776931,-12.1463643757414));
#83229=CARTESIAN_POINT('Ctrl Pts',(19.2888823973331,-16.9090046218179,-12.1467202324011));
#83230=CARTESIAN_POINT('Ctrl Pts',(19.3038343433411,-16.9131108835994,-12.1476430979305));
#83231=CARTESIAN_POINT('Ctrl Pts',(19.313016470345,-16.9156994476686,-12.1482088732589));
#83232=CARTESIAN_POINT('Ctrl Pts',(19.3442298136422,-16.9247271036667,-12.1501291029125));
#83233=CARTESIAN_POINT('Ctrl Pts',(19.366174156515,-16.9314625175157,-12.151473904434));
#83234=CARTESIAN_POINT('Ctrl Pts',(19.5553830930014,-16.99292114255,-12.1630344564364));
#83235=CARTESIAN_POINT('Ctrl Pts',(19.7153269906489,-17.0679447543458,-12.1724942695172));
#83236=CARTESIAN_POINT('Ctrl Pts',(19.9374236258115,-17.2081626030476,-12.1867867608847));
#83237=CARTESIAN_POINT('Ctrl Pts',(20.0077788230461,-17.2588719996558,-12.1915315574814));
#83238=CARTESIAN_POINT('Ctrl Pts',(20.1040235862784,-17.3376431034679,-12.1986330642438));
#83239=CARTESIAN_POINT('Ctrl Pts',(20.1325777323996,-17.3623167780314,-12.200825045838));
#83240=CARTESIAN_POINT('Ctrl Pts',(20.166046291059,-17.3928368676148,-12.203519995948));
#83241=CARTESIAN_POINT('Ctrl Pts',(20.1716098033111,-17.3979651539841,-12.2039722950571));
#83242=CARTESIAN_POINT('Ctrl Pts',(20.180204699436,-17.405973334838,-12.2046779931552));
#83243=CARTESIAN_POINT('Ctrl Pts',(20.1832553092452,-17.408832630596,-12.2049298433318));
#83244=CARTESIAN_POINT('Ctrl Pts',(20.1888904274041,-17.4141457983619,-12.2053976622854));
#83245=CARTESIAN_POINT('Ctrl Pts',(20.1914772173847,-17.416597166386,-12.2056134395859));
#83246=CARTESIAN_POINT('Ctrl Pts',(20.1973029608044,-17.4221459124098,-12.2061017116667));
#83247=CARTESIAN_POINT('Ctrl Pts',(20.2005382573396,-17.4252470326474,-12.2063744939988));
#83248=CARTESIAN_POINT('Ctrl Pts',(20.2100341785665,-17.4344071655437,-12.2071798626863));
#83249=CARTESIAN_POINT('Ctrl Pts',(20.2162671857352,-17.4404944950187,-12.2077145813135));
#83250=CARTESIAN_POINT('Ctrl Pts',(20.2603081210546,-17.4840404918751,-12.2115351001895));
#83251=CARTESIAN_POINT('Ctrl Pts',(20.2967260186452,-17.5228716087308,-12.2149175238978));
#83252=CARTESIAN_POINT('Ctrl Pts',(20.3436243467728,-17.5768155874372,-12.2195368360917));
#83253=CARTESIAN_POINT('Ctrl Pts',(20.3554306175602,-17.5907559249953,-12.2207238628777));
#83254=CARTESIAN_POINT('Ctrl Pts',(20.3976007705015,-17.6418757082568,-12.2250479487909));
#83255=CARTESIAN_POINT('Ctrl Pts',(20.426877799154,-17.6799317190139,-12.2282124605792));
#83256=CARTESIAN_POINT('Ctrl Pts',(20.5185421579863,-17.8078576836956,-12.2386083352236));
#83257=CARTESIAN_POINT('Ctrl Pts',(20.5752678670104,-17.9015770083348,-12.245840722962));
#83258=CARTESIAN_POINT('Ctrl Pts',(20.6492938150994,-18.0484658175535,-12.2564135071761));
#83259=CARTESIAN_POINT('Ctrl Pts',(20.6721600232126,-18.0986179271779,-12.2599022836881));
#83260=CARTESIAN_POINT('Ctrl Pts',(20.7060456980323,-18.1813500792953,-12.2654593465495));
#83261=CARTESIAN_POINT('Ctrl Pts',(20.7182736332477,-18.2134041023121,-12.2675660629028));
#83262=CARTESIAN_POINT('Ctrl Pts',(20.7333235416322,-18.2559316183104,-12.2703024289393));
#83263=CARTESIAN_POINT('Ctrl Pts',(20.736851244059,-18.2661481814058,-12.2709554164735));
#83264=CARTESIAN_POINT('Ctrl Pts',(20.7425019779367,-18.2829287135742,-12.2720208956252));
#83265=CARTESIAN_POINT('Ctrl Pts',(20.7446714096475,-18.2894767431454,-12.2724349165719));
#83266=CARTESIAN_POINT('Ctrl Pts',(20.7488094835661,-18.3021743043541,-12.2732344294919));
#83267=CARTESIAN_POINT('Ctrl Pts',(20.7507820698173,-18.3083224611045,-12.2736200477828));
#83268=CARTESIAN_POINT('Ctrl Pts',(20.7552726157238,-18.3225419026711,-12.2745084783195));
#83269=CARTESIAN_POINT('Ctrl Pts',(20.7577704237983,-18.33061947384,-12.2750106244516));
#83270=CARTESIAN_POINT('Ctrl Pts',(20.7643596515241,-18.3523893782569,-12.2763572728471));
#83271=CARTESIAN_POINT('Ctrl Pts',(20.7683609784959,-18.366108682152,-12.2771988334378));
#83272=CARTESIAN_POINT('Ctrl Pts',(20.803809115014,-18.4923927836866,-12.2848829072953));
#83273=CARTESIAN_POINT('Ctrl Pts',(20.8260248908665,-18.6073470023685,-12.2914085157882));
#83274=CARTESIAN_POINT('Ctrl Pts',(20.8562170107502,-18.885511157645,-12.3067257190411));
#83275=CARTESIAN_POINT('Ctrl Pts',(20.855041894869,-19.0489286551452,-12.3153337760523));
#83276=CARTESIAN_POINT('Ctrl Pts',(20.8312013426985,-19.2426549725124,-12.3265434425329));
#83277=CARTESIAN_POINT('Ctrl Pts',(20.8265193606268,-19.2746395096073,-12.3284289516276));
#83278=CARTESIAN_POINT('Ctrl Pts',(20.8198971723483,-19.3136271763478,-12.3307836283437));
#83279=CARTESIAN_POINT('Ctrl Pts',(20.8186505332077,-19.3207456837112,-12.3312158647962));
#83280=CARTESIAN_POINT('Ctrl Pts',(20.8166383401881,-19.3318992111781,-12.3318969324655));
#83281=CARTESIAN_POINT('Ctrl Pts',(20.8158974373662,-19.3359387012328,-12.3321443840855));
#83282=CARTESIAN_POINT('Ctrl Pts',(20.8144900990948,-19.3434878149372,-12.3326083465005));
#83283=CARTESIAN_POINT('Ctrl Pts',(20.813826532938,-19.3469979163289,-12.3328246929655));
#83284=CARTESIAN_POINT('Ctrl Pts',(20.8122908633305,-19.3550100698432,-12.3333199291672));
#83285=CARTESIAN_POINT('Ctrl Pts',(20.8114130169764,-19.3595109630199,-12.3335991422247));
#83286=CARTESIAN_POINT('Ctrl Pts',(20.8086674370288,-19.3733486567015,-12.3344605977594));
#83287=CARTESIAN_POINT('Ctrl Pts',(20.8067513590226,-19.3826755863278,-12.3350454933105));
#83288=CARTESIAN_POINT('Ctrl Pts',(20.7886241521695,-19.4679897984925,-12.3404326124482));
#83289=CARTESIAN_POINT('Ctrl Pts',(20.7683057282506,-19.5430358612127,-12.3454391348783));
#83290=CARTESIAN_POINT('Ctrl Pts',(20.7421027582796,-19.6222578030818,-12.3509004679087));
#83291=CARTESIAN_POINT('Ctrl Pts',(20.7402707671355,-19.6277217021486,-12.3512780632711));
#83292=CARTESIAN_POINT('Ctrl Pts',(20.6967115457058,-19.7558979180641,-12.3601569558555));
#83293=CARTESIAN_POINT('Ctrl Pts',(20.643820775992,-19.8745382004949,-12.3688045984896));
#83294=CARTESIAN_POINT('Ctrl Pts',(20.5373315123358,-20.0644025179968,-12.3828981078083));
#83295=CARTESIAN_POINT('Ctrl Pts',(20.4894988782859,-20.1384531113537,-12.388473695247));
#83296=CARTESIAN_POINT('Ctrl Pts',(20.4250114412864,-20.2258090596826,-12.3951372191672));
#83297=CARTESIAN_POINT('Ctrl Pts',(20.4125974797899,-20.2421239329334,-12.3963859637133));
#83298=CARTESIAN_POINT('Ctrl Pts',(20.3944831927711,-20.2652261840257,-12.3981608992562));
#83299=CARTESIAN_POINT('Ctrl Pts',(20.3889744822571,-20.2721616986906,-12.3986946352222));
#83300=CARTESIAN_POINT('Ctrl Pts',(20.3793483276385,-20.2841261647521,-12.3996169958875));
#83301=CARTESIAN_POINT('Ctrl Pts',(20.3752509819665,-20.289171063752,-12.4000064188428));
#83302=CARTESIAN_POINT('Ctrl Pts',(20.3673274996418,-20.298835646141,-12.4007534494684));
#83303=CARTESIAN_POINT('Ctrl Pts',(20.3635048390014,-20.3034580865175,-12.4011111922957));
#83304=CARTESIAN_POINT('Ctrl Pts',(20.3534377956224,-20.3155265525876,-12.4020464236606));
#83305=CARTESIAN_POINT('Ctrl Pts',(20.3471616531898,-20.3229459941818,-12.4026226113669));
#83306=CARTESIAN_POINT('Ctrl Pts',(20.3251950817667,-20.3485544114356,-12.4046158938871));
#83307=CARTESIAN_POINT('Ctrl Pts',(20.3092459722625,-20.3665197801725,-12.4060223004146));
#83308=CARTESIAN_POINT('Ctrl Pts',(20.1927900405548,-20.4932847509891,-12.4160147034109));
#83309=CARTESIAN_POINT('Ctrl Pts',(20.0814139780325,-20.5915454622472,-12.4240913569344));
#83310=CARTESIAN_POINT('Ctrl Pts',(19.92306194943,-20.704127586379,-12.4346429237359));
#83311=CARTESIAN_POINT('Ctrl Pts',(19.8845798500898,-20.7296347508308,-12.4371469729059));
#83312=CARTESIAN_POINT('Ctrl Pts',(19.7845284304216,-20.7913412476687,-12.443577247717));
#83313=CARTESIAN_POINT('Ctrl Pts',(19.7219089482267,-20.8257183800168,-12.4475276267364));
#83314=CARTESIAN_POINT('Ctrl Pts',(19.6274684418929,-20.8715130524845,-12.4535471089138));
#83315=CARTESIAN_POINT('Ctrl Pts',(19.5969164200343,-20.8854402450819,-12.455503677789));
#83316=CARTESIAN_POINT('Ctrl Pts',(19.5593254338195,-20.901507727772,-12.4579373746384));
#83317=CARTESIAN_POINT('Ctrl Pts',(19.5525879556011,-20.9043463339668,-12.4583745854735));
#83318=CARTESIAN_POINT('Ctrl Pts',(19.5420260195811,-20.9087319618677,-12.459061764027));
#83319=CARTESIAN_POINT('Ctrl Pts',(19.5382114393127,-20.9103028313123,-12.4593103109883));
#83320=CARTESIAN_POINT('Ctrl Pts',(19.5310874965847,-20.9132121930863,-12.4597752071622));
#83321=CARTESIAN_POINT('Ctrl Pts',(19.5277793318029,-20.9145534681338,-12.4599913851981));
#83322=CARTESIAN_POINT('Ctrl Pts',(19.5202392216401,-20.9175883760441,-12.4604847658428));
#83323=CARTESIAN_POINT('Ctrl Pts',(19.5160052057855,-20.9192767052226,-12.4607622823588));
#83324=CARTESIAN_POINT('Ctrl Pts',(19.5049829143421,-20.9236306785164,-12.4614858839157));
#83325=CARTESIAN_POINT('Ctrl Pts',(19.4981863242547,-20.9262749162593,-12.4619332043162));
#83326=CARTESIAN_POINT('Ctrl Pts',(19.4548256337707,-20.9428871005031,-12.4647935735592));
#83327=CARTESIAN_POINT('Ctrl Pts',(19.4178962004824,-20.9558728953422,-12.4672592521349));
#83328=CARTESIAN_POINT('Ctrl Pts',(19.3688752846647,-20.9715976798468,-12.4705516760663));
#83329=CARTESIAN_POINT('Ctrl Pts',(19.3570870694893,-20.9752656544818,-12.4713448815229));
#83330=CARTESIAN_POINT('Ctrl Pts',(19.3221513106599,-20.9858018597544,-12.4736986988017));
#83331=CARTESIAN_POINT('Ctrl Pts',(19.2989179826717,-20.9923773130897,-12.4752679913389));
#83332=CARTESIAN_POINT('Ctrl Pts',(19.1362196285474,-21.0354320514022,-12.4862637369298));
#83333=CARTESIAN_POINT('Ctrl Pts',(18.9934448152859,-21.0579827098367,-12.4959108586062));
#83334=CARTESIAN_POINT('Ctrl Pts',(18.787768864821,-21.069219491202,-12.5092191102238));
#83335=CARTESIAN_POINT('Ctrl Pts',(18.7259288608117,-21.0698870253441,-12.5131507017069));
#83336=CARTESIAN_POINT('Ctrl Pts',(18.6269048272022,-21.0666176610075,-12.519324324455));
#83337=CARTESIAN_POINT('Ctrl Pts',(18.5897034246201,-21.0644052649368,-12.5216162715323));
#83338=CARTESIAN_POINT('Ctrl Pts',(18.5414838674283,-21.0602576991223,-12.5245533668829));
#83339=CARTESIAN_POINT('Ctrl Pts',(18.5303974160802,-21.0592159316148,-12.5252263474334));
#83340=CARTESIAN_POINT('Ctrl Pts',(18.5123855121962,-21.0573799179716,-12.526316098293));
#83341=CARTESIAN_POINT('Ctrl Pts',(18.5054549621993,-21.0566388639639,-12.526734534482));
#83342=CARTESIAN_POINT('Ctrl Pts',(18.4921372980245,-21.0551483038057,-12.5275369584271));
#83343=CARTESIAN_POINT('Ctrl Pts',(18.4857497015159,-21.0544038967618,-12.5279211021013));
#83344=CARTESIAN_POINT('Ctrl Pts',(18.4711367121289,-21.052633380565,-12.5287982954899));
#83345=CARTESIAN_POINT('Ctrl Pts',(18.4629137220155,-21.0515880406703,-12.5292907332649));
#83346=CARTESIAN_POINT('Ctrl Pts',(18.4410945126435,-21.0486839725328,-12.53059438916));
#83347=CARTESIAN_POINT('Ctrl Pts',(18.4275097253491,-21.0467412799608,-12.5314029555338));
#83348=CARTESIAN_POINT('Ctrl Pts',(18.3247120750064,-21.0310192586882,-12.5374997932277));
#83349=CARTESIAN_POINT('Ctrl Pts',(18.2364379676942,-21.0116777835986,-12.5426055755362));
#83350=CARTESIAN_POINT('Ctrl Pts',(18.0155892361036,-20.9482545548448,-12.555325549663));
#83351=CARTESIAN_POINT('Ctrl Pts',(17.885658518111,-20.8965979403468,-12.5627450119146));
#83352=CARTESIAN_POINT('Ctrl Pts',(17.7126395596302,-20.8071466337983,-12.5735037478294));
#83353=CARTESIAN_POINT('Ctrl Pts',(17.6645406130502,-20.7798407894458,-12.5766018537881));
#83354=CARTESIAN_POINT('Ctrl Pts',(17.5933680194416,-20.73566449179,-12.5814337385233));
#83355=CARTESIAN_POINT('Ctrl Pts',(17.5694739215502,-20.7201569972724,-12.5831003841649));
#83356=CARTESIAN_POINT('Ctrl Pts',(17.5401543117035,-20.7002762041451,-12.5852110044489));
#83357=CARTESIAN_POINT('Ctrl Pts',(17.5344266223332,-20.6963511464121,-12.5856264965314));
#83358=CARTESIAN_POINT('Ctrl Pts',(17.5253935809179,-20.690095475009,-12.5862869789817));
#83359=CARTESIAN_POINT('Ctrl Pts',(17.5220753621259,-20.6877834046841,-12.586530724476));
#83360=CARTESIAN_POINT('Ctrl Pts',(17.5158296039964,-20.6834048421044,-12.5869916797798));
#83361=CARTESIAN_POINT('Ctrl Pts',(17.5129006790311,-20.6813404200953,-12.587208748946));
#83362=CARTESIAN_POINT('Ctrl Pts',(17.5062161289511,-20.6766034365492,-12.5877062175575));
#83363=CARTESIAN_POINT('Ctrl Pts',(17.5024639863758,-20.6739260418452,-12.5879869464144));
#83364=CARTESIAN_POINT('Ctrl Pts',(17.4925254501348,-20.6667851575629,-12.5887344346488));
#83365=CARTESIAN_POINT('Ctrl Pts',(17.4863544531645,-20.6623004940654,-12.5892025991234));
#83366=CARTESIAN_POINT('Ctrl Pts',(17.4432974653334,-20.6306525525968,-12.5924967344648));
#83367=CARTESIAN_POINT('Ctrl Pts',(17.4072802149826,-20.6023337083128,-12.595394769147));
#83368=CARTESIAN_POINT('Ctrl Pts',(17.3434298627298,-20.5486893666001,-12.6007562033481));
#83369=CARTESIAN_POINT('Ctrl Pts',(17.3152972309215,-20.5237456750931,-12.6032035622074));
#83370=CARTESIAN_POINT('Ctrl Pts',(17.1921807401655,-20.4085853896196,-12.6142536775164));
#83371=CARTESIAN_POINT('Ctrl Pts',(17.1050207763708,-20.3104101007053,-12.6229968788456));
#83372=CARTESIAN_POINT('Ctrl Pts',(16.9752027140399,-20.1335790198954,-12.6372013472694));
#83373=CARTESIAN_POINT('Ctrl Pts',(16.9274171686245,-20.0591399059462,-12.6427967463797));
#83374=CARTESIAN_POINT('Ctrl Pts',(16.8744284137836,-19.9639803676304,-12.6494812540878));
#83375=CARTESIAN_POINT('Ctrl Pts',(16.8646987212428,-19.9458931152881,-12.6507323074442));
#83376=CARTESIAN_POINT('Ctrl Pts',(16.8511486113747,-19.9198007064132,-12.6525099172039));
#83377=CARTESIAN_POINT('Ctrl Pts',(16.8471131304768,-19.9119091125399,-12.6530440498365));
#83378=CARTESIAN_POINT('Ctrl Pts',(16.8402042038597,-19.8981864167954,-12.6539668755691));
#83379=CARTESIAN_POINT('Ctrl Pts',(16.8373078570708,-19.8923670396287,-12.6543563691484));
#83380=CARTESIAN_POINT('Ctrl Pts',(16.8317911218727,-19.881153563582,-12.6551033824457));
#83381=CARTESIAN_POINT('Ctrl Pts',(16.8291667639058,-19.8757614976569,-12.6554610380493));
#83382=CARTESIAN_POINT('Ctrl Pts',(16.8223533114919,-19.8616099239209,-12.6563957027042));
#83383=CARTESIAN_POINT('Ctrl Pts',(16.818201475293,-19.8528325554072,-12.6569714140286));
#83384=CARTESIAN_POINT('Ctrl Pts',(16.8040088662289,-19.8222861123193,-12.6589613888741));
#83385=CARTESIAN_POINT('Ctrl Pts',(16.7942773404032,-19.8003747794809,-12.6603650119482));
#83386=CARTESIAN_POINT('Ctrl Pts',(16.7708981679383,-19.7452280274813,-12.6638421844087));
#83387=CARTESIAN_POINT('Ctrl Pts',(16.7577281088485,-19.7118198611918,-12.6658990953057));
#83388=CARTESIAN_POINT('Ctrl Pts',(16.7454195349593,-19.6781106899492,-12.6679318731853));
#83389=CARTESIAN_POINT('',(16.6141771461173,-18.9509225630941,-11.6890562790225));
#83390=CARTESIAN_POINT('Ctrl Pts',(16.7437496527793,-19.6787359237804,-12.4443820746906));
#83391=CARTESIAN_POINT('Ctrl Pts',(16.9543734450167,-20.2394180692954,-12.4082724658268));
#83392=CARTESIAN_POINT('Ctrl Pts',(17.9482901965323,-21.2712729007906,-12.3297709214024));
#83393=CARTESIAN_POINT('Ctrl Pts',(20.2082246479652,-20.9751142883798,-12.2088774414178));
#83394=CARTESIAN_POINT('Ctrl Pts',(21.2330887928116,-18.8074837650725,-12.0817016347363));
#83395=CARTESIAN_POINT('Ctrl Pts',(19.9651940811972,-16.7724379176221,-11.9545258280548));
#83396=CARTESIAN_POINT('Ctrl Pts',(17.5677552166072,-16.7370050018739,-11.8273500213735));
#83397=CARTESIAN_POINT('Ctrl Pts',(16.6440838383059,-18.1263146735576,-11.7388601716959));
#83398=CARTESIAN_POINT('Ctrl Pts',(16.6137960417384,-18.8895339291486,-11.692762257579));
#83399=CARTESIAN_POINT('Ctrl Pts',(16.6141771461173,-18.9509225630941,-11.6890562790225));
#83400=CARTESIAN_POINT('Ctrl Pts',(16.6170002227512,-18.951028851869,-11.6906772973237));
#83401=CARTESIAN_POINT('Ctrl Pts',(16.6169204646911,-19.1248929515366,-11.6794936821839));
#83402=CARTESIAN_POINT('Ctrl Pts',(16.6382580402862,-19.2981155640509,-11.66776312738));
#83403=CARTESIAN_POINT('Ctrl Pts',(16.6953875256918,-19.5259976394338,-11.6525929584797));
#83404=CARTESIAN_POINT('Ctrl Pts',(16.7127834335452,-19.5845336305672,-11.648712703421));
#83405=CARTESIAN_POINT('Ctrl Pts',(16.7368231144309,-19.6542353438915,-11.6441197397871));
#83406=CARTESIAN_POINT('Ctrl Pts',(16.7410677156335,-19.666192471166,-11.6433327722891));
#83407=CARTESIAN_POINT('Ctrl Pts',(16.7454194494007,-19.678110455632,-11.6425492951846));
#83408=CARTESIAN_POINT('Origin',(18.734,-18.952,0.));
#83409=CARTESIAN_POINT('',(16.7454194496957,-19.67811045644,-10.8441190240937));
#83410=CARTESIAN_POINT('',(16.745419450227,-19.678110457895,-11.0644158965713));
#83411=CARTESIAN_POINT('',(16.7454194499637,-19.6781104571739,0.));
#83412=CARTESIAN_POINT('Ctrl Pts',(16.745419450227,-19.678110457895,-11.0644158965713));
#83413=CARTESIAN_POINT('Ctrl Pts',(16.7100155218545,-19.581150604774,-11.0708124074204));
#83414=CARTESIAN_POINT('Ctrl Pts',(16.6817531145212,-19.4817385259306,-11.0775606813504));
#83415=CARTESIAN_POINT('Ctrl Pts',(16.6317924848945,-19.2401187266275,-11.0938351403994));
#83416=CARTESIAN_POINT('Ctrl Pts',(16.6170952308914,-19.0969558973671,-11.1033537401525));
#83417=CARTESIAN_POINT('Ctrl Pts',(16.6169595358669,-18.8914033897129,-11.1164063607099));
#83418=CARTESIAN_POINT('Ctrl Pts',(16.6196417425704,-18.8294329463025,-11.1202674028607));
#83419=CARTESIAN_POINT('Ctrl Pts',(16.626121995978,-18.755293290851,-11.1248001906107));
#83420=CARTESIAN_POINT('Ctrl Pts',(16.6273121369964,-18.7429319071468,-11.125553102198));
#83421=CARTESIAN_POINT('Ctrl Pts',(16.629446086491,-18.7226409476578,-11.126784473422));
#83422=CARTESIAN_POINT('Ctrl Pts',(16.6303260988315,-18.7147050990314,-11.12726492884));
#83423=CARTESIAN_POINT('Ctrl Pts',(16.6319896971568,-18.7004401578214,-11.1281265731885));
#83424=CARTESIAN_POINT('Ctrl Pts',(16.6327570212934,-18.6941092997592,-11.1285082696425));
#83425=CARTESIAN_POINT('Ctrl Pts',(16.6344530088088,-18.6806267538166,-11.1293196853172));
#83426=CARTESIAN_POINT('Ctrl Pts',(16.6353896346168,-18.6734761352318,-11.1297491481872));
#83427=CARTESIAN_POINT('Ctrl Pts',(16.6380125558554,-18.6542163446122,-11.1309035864619));
#83428=CARTESIAN_POINT('Ctrl Pts',(16.6397672552717,-18.6421166480973,-11.1316263951854));
#83429=CARTESIAN_POINT('Ctrl Pts',(16.6490971421965,-18.5814843962378,-11.1352369299879));
#83430=CARTESIAN_POINT('Ctrl Pts',(16.6582553372663,-18.5332084216257,-11.1380741371182));
#83431=CARTESIAN_POINT('Ctrl Pts',(16.6895710826044,-18.3946543047097,-11.1461497795195));
#83432=CARTESIAN_POINT('Ctrl Pts',(16.7160033266981,-18.30545898715,-11.1512603837602));
#83433=CARTESIAN_POINT('Ctrl Pts',(16.8056500674886,-18.0628317947687,-11.1653489073645));
#83434=CARTESIAN_POINT('Ctrl Pts',(16.8811330566578,-17.9146858719793,-11.1741493553049));
#83435=CARTESIAN_POINT('Ctrl Pts',(16.9808578003806,-17.7652494132739,-11.1847107322291));
#83436=CARTESIAN_POINT('Ctrl Pts',(16.9887344573945,-17.7536959110232,-11.185539392666));
#83437=CARTESIAN_POINT('Ctrl Pts',(16.9998805495105,-17.7376898139786,-11.186705694803));
#83438=CARTESIAN_POINT('Ctrl Pts',(17.0030540299258,-17.733170420623,-11.1870370642763));
#83439=CARTESIAN_POINT('Ctrl Pts',(17.0081863112416,-17.7259219452459,-11.1875719448114));
#83440=CARTESIAN_POINT('Ctrl Pts',(17.0101340136098,-17.7231849833039,-11.1877746979201));
#83441=CARTESIAN_POINT('Ctrl Pts',(17.0142251822704,-17.7174648363681,-11.1882001205937));
#83442=CARTESIAN_POINT('Ctrl Pts',(17.0163699008623,-17.7144825917355,-11.1884228794976));
#83443=CARTESIAN_POINT('Ctrl Pts',(17.0215923833771,-17.7072604270757,-11.1889646472359));
#83444=CARTESIAN_POINT('Ctrl Pts',(17.0246781354636,-17.703026336571,-11.1892842039935));
#83445=CARTESIAN_POINT('Ctrl Pts',(17.035608726877,-17.6881443901401,-11.1904140998444));
#83446=CARTESIAN_POINT('Ctrl Pts',(17.0435374121948,-17.6775588918596,-11.191229976263));
#83447=CARTESIAN_POINT('Ctrl Pts',(17.0915650943686,-17.6146744264093,-11.1961467226523));
#83448=CARTESIAN_POINT('Ctrl Pts',(17.1339858171065,-17.5642013661841,-11.2003844556965));
#83449=CARTESIAN_POINT('Ctrl Pts',(17.2439182099723,-17.4451520632016,-11.2109620933829));
#83450=CARTESIAN_POINT('Ctrl Pts',(17.3138862301183,-17.3790374597029,-11.2173577648922));
#83451=CARTESIAN_POINT('Ctrl Pts',(17.4967378723479,-17.2284345152286,-11.2329413052017));
#83452=CARTESIAN_POINT('Ctrl Pts',(17.6140381009902,-17.1500027268374,-11.2419898436872));
#83453=CARTESIAN_POINT('Ctrl Pts',(17.7508858952365,-17.0770653821329,-11.2514584928521));
#83454=CARTESIAN_POINT('Ctrl Pts',(17.7635632824206,-17.0704724936505,-11.252326423371));
#83455=CARTESIAN_POINT('Ctrl Pts',(17.783846444058,-17.0601837575227,-11.2537006737471));
#83456=CARTESIAN_POINT('Ctrl Pts',(17.791409118207,-17.0564043395359,-11.2542099212861));
#83457=CARTESIAN_POINT('Ctrl Pts',(17.804787123036,-17.049818589606,-11.2551052842454));
#83458=CARTESIAN_POINT('Ctrl Pts',(17.8105929943291,-17.0469933879183,-11.2554920557224));
#83459=CARTESIAN_POINT('Ctrl Pts',(17.8226282444429,-17.0412048493931,-11.2562901274364));
#83460=CARTESIAN_POINT('Ctrl Pts',(17.8288593707787,-17.0382453063481,-11.256701292256));
#83461=CARTESIAN_POINT('Ctrl Pts',(17.8448911760841,-17.0307266371575,-11.2577540305011));
#83462=CARTESIAN_POINT('Ctrl Pts',(17.8547125844484,-17.0262119839024,-11.2583940624616));
#83463=CARTESIAN_POINT('Ctrl Pts',(17.8958499793224,-17.0076824792482,-11.2610549526072));
#83464=CARTESIAN_POINT('Ctrl Pts',(17.9274707769542,-16.9943542486712,-11.2630522769814));
#83465=CARTESIAN_POINT('Ctrl Pts',(18.0106938754143,-16.9616345434039,-11.2681969743295));
#83466=CARTESIAN_POINT('Ctrl Pts',(18.0627550143649,-16.9434788486161,-11.2713049458654));
#83467=CARTESIAN_POINT('Ctrl Pts',(18.2200495552602,-16.8954247017299,-11.2804500761598));
#83468=CARTESIAN_POINT('Ctrl Pts',(18.3269519425295,-16.8716250869388,-11.2863385079318));
#83469=CARTESIAN_POINT('Ctrl Pts',(18.481091160126,-16.8496504561494,-11.2948153762593));
#83470=CARTESIAN_POINT('Ctrl Pts',(18.5271693679278,-16.8446183718685,-11.2973493544173));
#83471=CARTESIAN_POINT('Ctrl Pts',(18.5947046835901,-16.8394793624749,-11.3011064816897));
#83472=CARTESIAN_POINT('Ctrl Pts',(18.616058174059,-16.8381796878557,-11.3023007363443));
#83473=CARTESIAN_POINT('Ctrl Pts',(18.689228025621,-16.8348383636923,-11.3064251625996));
#83474=CARTESIAN_POINT('Ctrl Pts',(18.7410938586039,-16.8343771210788,-11.3094038306521));
#83475=CARTESIAN_POINT('Ctrl Pts',(18.8015714509149,-16.8360609618551,-11.3129946089349));
#83476=CARTESIAN_POINT('Ctrl Pts',(18.8102216668728,-16.8363549055115,-11.3135110167586));
#83477=CARTESIAN_POINT('Ctrl Pts',(18.8233353012831,-16.8368810487547,-11.314298477698));
#83478=CARTESIAN_POINT('Ctrl Pts',(18.8278003077781,-16.8370743570067,-11.3145674047013));
#83479=CARTESIAN_POINT('Ctrl Pts',(18.8358238711881,-16.8374471879692,-11.3150521684942));
#83480=CARTESIAN_POINT('Ctrl Pts',(18.8393826131848,-16.8376215570191,-11.3152677139316));
#83481=CARTESIAN_POINT('Ctrl Pts',(18.8471261343323,-16.8380205677217,-11.3157378982348));
#83482=CARTESIAN_POINT('Ctrl Pts',(18.851310637997,-16.838248648522,-11.3159927223016));
#83483=CARTESIAN_POINT('Ctrl Pts',(18.8630926444103,-16.8389259328327,-11.3167122498838));
#83484=CARTESIAN_POINT('Ctrl Pts',(18.8706883516572,-16.8394036791997,-11.3171785070507));
#83485=CARTESIAN_POINT('Ctrl Pts',(18.9167070206829,-16.8425473269248,-11.3200171271687));
#83486=CARTESIAN_POINT('Ctrl Pts',(18.9550513628164,-16.8462202633494,-11.3224405987897));
#83487=CARTESIAN_POINT('Ctrl Pts',(19.0823659376831,-16.8619308840319,-11.3306355105033));
#83488=CARTESIAN_POINT('Ctrl Pts',(19.1706657035548,-16.8785804052242,-11.336558067772));
#83489=CARTESIAN_POINT('Ctrl Pts',(19.4238492837337,-16.943213248176,-11.3538251334834));
#83490=CARTESIAN_POINT('Ctrl Pts',(19.5843224133701,-17.0056983747675,-11.3650716078246));
#83491=CARTESIAN_POINT('Ctrl Pts',(19.7560025096065,-17.0978854440289,-11.3770690612865));
#83492=CARTESIAN_POINT('Ctrl Pts',(19.7763108052372,-17.1092254154925,-11.3784891007252));
#83493=CARTESIAN_POINT('Ctrl Pts',(19.8047237132041,-17.1257109485089,-11.38047776238));
#83494=CARTESIAN_POINT('Ctrl Pts',(19.8129859695544,-17.1305801549745,-11.3810562864926));
#83495=CARTESIAN_POINT('Ctrl Pts',(19.8263416371281,-17.1385738377566,-11.3819919211739));
#83496=CARTESIAN_POINT('Ctrl Pts',(19.8314553405053,-17.1416639884136,-11.3823502758451));
#83497=CARTESIAN_POINT('Ctrl Pts',(19.8421198935967,-17.1481702459721,-11.3830978859057));
#83498=CARTESIAN_POINT('Ctrl Pts',(19.8476681945754,-17.1515904260537,-11.3834869868843));
#83499=CARTESIAN_POINT('Ctrl Pts',(19.8608077281338,-17.159774104919,-11.384408870361));
#83500=CARTESIAN_POINT('Ctrl Pts',(19.8683847211791,-17.1645603161789,-11.384940808165));
#83501=CARTESIAN_POINT('Ctrl Pts',(19.8937059951239,-17.1807810409493,-11.3867197769175));
#83502=CARTESIAN_POINT('Ctrl Pts',(19.9113099570464,-17.1924330338004,-11.3879587111698));
#83503=CARTESIAN_POINT('Ctrl Pts',(20.0055405439043,-17.2568512942767,-11.3946073015226));
#83504=CARTESIAN_POINT('Ctrl Pts',(20.0788040825999,-17.3143647018779,-11.3998313584646));
#83505=CARTESIAN_POINT('Ctrl Pts',(20.2632223604968,-17.4798868380565,-11.4134779554991));
#83506=CARTESIAN_POINT('Ctrl Pts',(20.3667005746358,-17.5955632781556,-11.4216615554222));
#83507=CARTESIAN_POINT('Ctrl Pts',(20.4878034878973,-17.7650979442364,-11.4333758771198));
#83508=CARTESIAN_POINT('Ctrl Pts',(20.5172944170812,-17.8098865409465,-11.4364515234528));
#83509=CARTESIAN_POINT('Ctrl Pts',(20.5495766267374,-17.8632177062726,-11.4401508612578));
#83510=CARTESIAN_POINT('Ctrl Pts',(20.5540555868417,-17.8707215781585,-11.440672201567));
#83511=CARTESIAN_POINT('Ctrl Pts',(20.5607638284928,-17.8821200765634,-11.441465714825));
#83512=CARTESIAN_POINT('Ctrl Pts',(20.5630274603093,-17.8859945195991,-11.441735712348));
#83513=CARTESIAN_POINT('Ctrl Pts',(20.5670669568691,-17.8929592852595,-11.4422216125198));
#83514=CARTESIAN_POINT('Ctrl Pts',(20.5688473494059,-17.896046919637,-11.442437217712));
#83515=CARTESIAN_POINT('Ctrl Pts',(20.5726972193058,-17.9027626669011,-11.442906603626));
#83516=CARTESIAN_POINT('Ctrl Pts',(20.5747637321573,-17.9063923646366,-11.4431605644725));
#83517=CARTESIAN_POINT('Ctrl Pts',(20.5805337598745,-17.9165971691968,-11.4438752712907));
#83518=CARTESIAN_POINT('Ctrl Pts',(20.5842128351908,-17.9231859210976,-11.4443375384607));
#83519=CARTESIAN_POINT('Ctrl Pts',(20.6059073569254,-17.9625307639731,-11.4471021682087));
#83520=CARTESIAN_POINT('Ctrl Pts',(20.6230866320162,-17.995737576871,-11.4494526570944));
#83521=CARTESIAN_POINT('Ctrl Pts',(20.6765427211136,-18.1061339463082,-11.4572808214052));
#83522=CARTESIAN_POINT('Ctrl Pts',(20.7090346744814,-18.1850594753952,-11.462896260796));
#83523=CARTESIAN_POINT('Ctrl Pts',(20.7943566477514,-18.4340440717106,-11.480283677724));
#83524=CARTESIAN_POINT('Ctrl Pts',(20.830598246833,-18.6090013489265,-11.4919758281924));
#83525=CARTESIAN_POINT('Ctrl Pts',(20.846300249462,-18.8091838028158,-11.5043329499581));
#83526=CARTESIAN_POINT('Ctrl Pts',(20.847715871368,-18.8319413102655,-11.5057246001045));
#83527=CARTESIAN_POINT('Ctrl Pts',(20.8492008518456,-18.8642225299582,-11.5076806946153));
#83528=CARTESIAN_POINT('Ctrl Pts',(20.849573999591,-18.8737300519176,-11.5082546080407));
#83529=CARTESIAN_POINT('Ctrl Pts',(20.8500766583254,-18.8891978439929,-11.5091848146042));
#83530=CARTESIAN_POINT('Ctrl Pts',(20.8502451105319,-18.8951566363744,-11.5095423235335));
#83531=CARTESIAN_POINT('Ctrl Pts',(20.8505453361092,-18.9076437695096,-11.5102897769738));
#83532=CARTESIAN_POINT('Ctrl Pts',(20.8506720795346,-18.9141721771657,-11.5106795600102));
#83533=CARTESIAN_POINT('Ctrl Pts',(20.8509020826932,-18.9297274789792,-11.5116059820139));
#83534=CARTESIAN_POINT('Ctrl Pts',(20.8509778125364,-18.9387546998574,-11.5121417535886));
#83535=CARTESIAN_POINT('Ctrl Pts',(20.8510386248689,-18.9692778580766,-11.5139472425122));
#83536=CARTESIAN_POINT('Ctrl Pts',(20.8507540561398,-18.9907734375804,-11.5152085244988));
#83537=CARTESIAN_POINT('Ctrl Pts',(20.8450325209335,-19.1916906175374,-11.5269113883742));
#83538=CARTESIAN_POINT('Ctrl Pts',(20.8171253807949,-19.3697385869319,-11.5365557069102));
#83539=CARTESIAN_POINT('Ctrl Pts',(20.7335064491919,-19.6578110194735,-11.5528807639419));
#83540=CARTESIAN_POINT('Ctrl Pts',(20.6901264942475,-19.7703861615986,-11.5594887378648));
#83541=CARTESIAN_POINT('Ctrl Pts',(20.6332651972428,-19.8871849646391,-11.5671876724371));
#83542=CARTESIAN_POINT('Ctrl Pts',(20.6290505370366,-19.8956962763619,-11.567753802325));
#83543=CARTESIAN_POINT('Ctrl Pts',(20.6227183965027,-19.9082702570294,-11.5685981618811));
#83544=CARTESIAN_POINT('Ctrl Pts',(20.6206447032474,-19.9123550117381,-11.5688737186914));
#83545=CARTESIAN_POINT('Ctrl Pts',(20.6169305648842,-19.9196126529449,-11.5693656209368));
#83546=CARTESIAN_POINT('Ctrl Pts',(20.6152953318631,-19.9227881501101,-11.5695816373332));
#83547=CARTESIAN_POINT('Ctrl Pts',(20.6117611639355,-19.9296087681366,-11.5700473343768));
#83548=CARTESIAN_POINT('Ctrl Pts',(20.6098596759973,-19.9332524484686,-11.5702971705856));
#83549=CARTESIAN_POINT('Ctrl Pts',(20.6045788323012,-19.9433002904242,-11.5709889862551));
#83550=CARTESIAN_POINT('Ctrl Pts',(20.6011772477073,-19.9496926158906,-11.571432337035));
#83551=CARTESIAN_POINT('Ctrl Pts',(20.5823143017834,-19.9847058911838,-11.5738779785628));
#83552=CARTESIAN_POINT('Ctrl Pts',(20.5662285129147,-20.0129833284871,-11.5759165958648));
#83553=CARTESIAN_POINT('Ctrl Pts',(20.4658095905838,-20.1804130868523,-11.5883224672041));
#83554=CARTESIAN_POINT('Ctrl Pts',(20.3663158597173,-20.3098321079309,-11.5992797311881));
#83555=CARTESIAN_POINT('Ctrl Pts',(20.1716352093816,-20.5103752205316,-11.6175362417707));
#83556=CARTESIAN_POINT('Ctrl Pts',(20.0834833576251,-20.5873075526402,-11.6249755958214));
#83557=CARTESIAN_POINT('Ctrl Pts',(19.9779040037503,-20.6650663736084,-11.6329821437773));
#83558=CARTESIAN_POINT('Ctrl Pts',(19.9663016505822,-20.6734314475657,-11.6338509499323));
#83559=CARTESIAN_POINT('Ctrl Pts',(19.9477042969118,-20.6865553967925,-11.63522632025));
#83560=CARTESIAN_POINT('Ctrl Pts',(19.9407641663374,-20.6913909264373,-11.6357358195233));
#83561=CARTESIAN_POINT('Ctrl Pts',(19.9284749774271,-20.6998444512602,-11.6366314753259));
#83562=CARTESIAN_POINT('Ctrl Pts',(19.9231380320171,-20.7034797857082,-11.6370182892629));
#83563=CARTESIAN_POINT('Ctrl Pts',(19.9120669961836,-20.7109470469126,-11.6378163052585));
#83564=CARTESIAN_POINT('Ctrl Pts',(19.9063306407073,-20.7147754910734,-11.6382273726062));
#83565=CARTESIAN_POINT('Ctrl Pts',(19.8915621430436,-20.7245280127199,-11.6392795647702));
#83566=CARTESIAN_POINT('Ctrl Pts',(19.8825031142347,-20.730411165626,-11.6399191512599));
#83567=CARTESIAN_POINT('Ctrl Pts',(19.8445396250015,-20.7546545086083,-11.6425757148039));
#83568=CARTESIAN_POINT('Ctrl Pts',(19.8152359218099,-20.7723819964638,-11.6445692556177));
#83569=CARTESIAN_POINT('Ctrl Pts',(19.7378073837054,-20.8166932775471,-11.6497020092391));
#83570=CARTESIAN_POINT('Ctrl Pts',(19.6890536395695,-20.8421278977151,-11.6528020600797));
#83571=CARTESIAN_POINT('Ctrl Pts',(19.4687993257244,-20.9463325689024,-11.6663519919665));
#83572=CARTESIAN_POINT('Ctrl Pts',(19.2882366847939,-21.0038528895329,-11.6761989408021));
#83573=CARTESIAN_POINT('Ctrl Pts',(19.0615074184092,-21.0439268018128,-11.6892860114667));
#83574=CARTESIAN_POINT('Ctrl Pts',(19.0203493023044,-21.0499567236923,-11.6916931577766));
#83575=CARTESIAN_POINT('Ctrl Pts',(18.9716775158194,-21.0556286253397,-11.6946045340791));
#83576=CARTESIAN_POINT('Ctrl Pts',(18.9643071724426,-21.0564482881614,-11.6950471458896));
#83577=CARTESIAN_POINT('Ctrl Pts',(18.9523629445168,-21.0577131196342,-11.6957674754418));
#83578=CARTESIAN_POINT('Ctrl Pts',(18.9477915774475,-21.0581821569458,-11.6960438851429));
#83579=CARTESIAN_POINT('Ctrl Pts',(18.9396629915502,-21.0589894404498,-11.6965367218354));
#83580=CARTESIAN_POINT('Ctrl Pts',(18.9361064069539,-21.0593335683528,-11.6967528149547));
#83581=CARTESIAN_POINT('Ctrl Pts',(18.9284664178618,-21.060053278984,-11.6972180080085));
#83582=CARTESIAN_POINT('Ctrl Pts',(18.9243828489696,-21.0604259970107,-11.6974672599795));
#83583=CARTESIAN_POINT('Ctrl Pts',(18.9131280453586,-21.0614202892363,-11.6981558507593));
#83584=CARTESIAN_POINT('Ctrl Pts',(18.9059547614629,-21.0620171491854,-11.6985965403282));
#83585=CARTESIAN_POINT('Ctrl Pts',(18.866967454166,-21.0650609975284,-11.7010010584365));
#83586=CARTESIAN_POINT('Ctrl Pts',(18.8351060686448,-21.0668249173981,-11.7029998170707));
#83587=CARTESIAN_POINT('Ctrl Pts',(18.640068020497,-21.0732054446071,-11.7153925258526));
#83588=CARTESIAN_POINT('Ctrl Pts',(18.4768518915982,-21.0596552023776,-11.7263866294886));
#83589=CARTESIAN_POINT('Ctrl Pts',(18.20214747427,-21.0044380104952,-11.7446901734978));
#83590=CARTESIAN_POINT('Ctrl Pts',(18.0895730541209,-20.9719234247227,-11.752141069334));
#83591=CARTESIAN_POINT('Ctrl Pts',(17.9668806515865,-20.9251754744995,-11.760158164));
#83592=CARTESIAN_POINT('Ctrl Pts',(17.9535675725374,-20.9199478625717,-11.7610269205312));
#83593=CARTESIAN_POINT('Ctrl Pts',(17.9324669848438,-20.9114145468859,-11.7624022273827));
#83594=CARTESIAN_POINT('Ctrl Pts',(17.9246447269608,-20.908196458994,-11.7629117123923));
#83595=CARTESIAN_POINT('Ctrl Pts',(17.9108849996322,-20.9024390257515,-11.7638073516));
#83596=CARTESIAN_POINT('Ctrl Pts',(17.904939508024,-20.8999192486042,-11.764194163129));
#83597=CARTESIAN_POINT('Ctrl Pts',(17.89353031424,-20.895022184358,-11.7649361137698));
#83598=CARTESIAN_POINT('Ctrl Pts',(17.8880649449864,-20.8926489598597,-11.7652913866667));
#83599=CARTESIAN_POINT('Ctrl Pts',(17.8736608268599,-20.8863218551937,-11.7662273757033));
#83600=CARTESIAN_POINT('Ctrl Pts',(17.8647392476091,-20.8823290604288,-11.7668067564509));
#83601=CARTESIAN_POINT('Ctrl Pts',(17.8317010607084,-20.8672675359174,-11.7689512987458));
#83602=CARTESIAN_POINT('Ctrl Pts',(17.8077649311691,-20.8558071856561,-11.7705029736344));
#83603=CARTESIAN_POINT('Ctrl Pts',(17.748947324973,-20.8262740102284,-11.7743156114004));
#83604=CARTESIAN_POINT('Ctrl Pts',(17.714340864297,-20.8076743647222,-11.7765585129559));
#83605=CARTESIAN_POINT('Ctrl Pts',(17.5863822921762,-20.7342403812065,-11.7848824047792));
#83606=CARTESIAN_POINT('Ctrl Pts',(17.4967606950483,-20.6732345109063,-11.7907660949882));
#83607=CARTESIAN_POINT('Ctrl Pts',(17.3058049119968,-20.5205977406213,-11.8040416219604));
#83608=CARTESIAN_POINT('Ctrl Pts',(17.2078836688361,-20.4254988128732,-11.8113988900472));
#83609=CARTESIAN_POINT('Ctrl Pts',(17.1096883063368,-20.309771757951,-11.8202986764722));
#83610=CARTESIAN_POINT('Ctrl Pts',(17.0997220685116,-20.2977593527334,-11.8212220650879));
#83611=CARTESIAN_POINT('Ctrl Pts',(17.0862500243317,-20.2811510078491,-11.8224999238372));
#83612=CARTESIAN_POINT('Ctrl Pts',(17.0826285854063,-20.276648947179,-11.8228464330432));
#83613=CARTESIAN_POINT('Ctrl Pts',(17.0769000682388,-20.2694674323153,-11.8233994590358));
#83614=CARTESIAN_POINT('Ctrl Pts',(17.0747809226385,-20.2667975783345,-11.8236051189291));
#83615=CARTESIAN_POINT('Ctrl Pts',(17.0704149017473,-20.2612695820176,-11.8240310993708));
#83616=CARTESIAN_POINT('Ctrl Pts',(17.0681689443871,-20.2584107741834,-11.8242514848359));
#83617=CARTESIAN_POINT('Ctrl Pts',(17.0628304826103,-20.2515794661267,-11.8247782984213));
#83618=CARTESIAN_POINT('Ctrl Pts',(17.0597447725791,-20.2476017045694,-11.8250852033133));
#83619=CARTESIAN_POINT('Ctrl Pts',(17.049365876814,-20.2341233650724,-11.8261255221791));
#83620=CARTESIAN_POINT('Ctrl Pts',(17.0421392933951,-20.22457211446,-11.8268633902977));
#83621=CARTESIAN_POINT('Ctrl Pts',(16.9597880278116,-20.1137885334449,-11.8354244059807));
#83622=CARTESIAN_POINT('Ctrl Pts',(16.8937766098522,-20.0061119203458,-11.8437552230649));
#83623=CARTESIAN_POINT('Ctrl Pts',(16.8040373496761,-19.8253154296891,-11.8570939438366));
#83624=CARTESIAN_POINT('Ctrl Pts',(16.7740037979316,-19.7556488786253,-11.8620971149624));
#83625=CARTESIAN_POINT('Ctrl Pts',(16.746983787129,-19.6823839726103,-11.8671696135929));
#83626=CARTESIAN_POINT('Ctrl Pts',(16.7461998923975,-19.680247835349,-11.8673173497811));
#83627=CARTESIAN_POINT('Ctrl Pts',(16.7454194500115,-19.678110457305,-11.8674650116542));
#83628=CARTESIAN_POINT('Ctrl Pts',(16.7454194494007,-19.678110455632,-11.6425492951846));
#83629=CARTESIAN_POINT('Ctrl Pts',(16.7537320415196,-19.7008759438364,-11.641052713373));
#83630=CARTESIAN_POINT('Ctrl Pts',(16.7624355372938,-19.7234986099059,-11.6395688907372));
#83631=CARTESIAN_POINT('Ctrl Pts',(16.7756890193127,-19.7562576066727,-11.6374244257199));
#83632=CARTESIAN_POINT('Ctrl Pts',(16.7799326697562,-19.7665140092076,-11.6367536253212));
#83633=CARTESIAN_POINT('Ctrl Pts',(16.7869691239472,-19.7831487461488,-11.6356665220664));
#83634=CARTESIAN_POINT('Ctrl Pts',(16.7897130352974,-19.7895474143097,-11.6352485684289));
#83635=CARTESIAN_POINT('Ctrl Pts',(16.7950530958861,-19.8018325072886,-11.6344464789995));
#83636=CARTESIAN_POINT('Ctrl Pts',(16.7976446063523,-19.8077208530353,-11.6340621904555));
#83637=CARTESIAN_POINT('Ctrl Pts',(16.8036434320464,-19.8211843944791,-11.6331838465548));
#83638=CARTESIAN_POINT('Ctrl Pts',(16.8070685823025,-19.8287515643208,-11.6326904086965));
#83639=CARTESIAN_POINT('Ctrl Pts',(16.8162945366403,-19.8488191900349,-11.6313823452923));
#83640=CARTESIAN_POINT('Ctrl Pts',(16.8221730716316,-19.8612836263645,-11.6305704005356));
#83641=CARTESIAN_POINT('Ctrl Pts',(16.8684507528882,-19.956974427592,-11.6243391614861));
#83642=CARTESIAN_POINT('Ctrl Pts',(16.9141469455404,-20.0375346612341,-11.6191121174511));
#83643=CARTESIAN_POINT('Ctrl Pts',(17.0421776798662,-20.2323052295042,-11.6062233171191));
#83644=CARTESIAN_POINT('Ctrl Pts',(17.1308833385095,-20.3417693801885,-11.5987519067365));
#83645=CARTESIAN_POINT('Ctrl Pts',(17.2669684822215,-20.4791872697837,-11.5880489464911));
#83646=CARTESIAN_POINT('Ctrl Pts',(17.3055494660927,-20.5153332152072,-11.585081337342));
#83647=CARTESIAN_POINT('Ctrl Pts',(17.3592981732938,-20.5620375674297,-11.5809699964668));
#83648=CARTESIAN_POINT('Ctrl Pts',(17.3733124438585,-20.5738987049384,-11.579899980928));
#83649=CARTESIAN_POINT('Ctrl Pts',(17.3942413803745,-20.5911499772119,-11.5783018611282));
#83650=CARTESIAN_POINT('Ctrl Pts',(17.4010384686044,-20.5966821445999,-11.5777828157609));
#83651=CARTESIAN_POINT('Ctrl Pts',(17.4133462435462,-20.6065730627821,-11.5768425119513));
#83652=CARTESIAN_POINT('Ctrl Pts',(17.4188446926063,-20.6109469186219,-11.5764222765148));
#83653=CARTESIAN_POINT('Ctrl Pts',(17.4275603138112,-20.6178093795621,-11.5757557276745));
#83654=CARTESIAN_POINT('Ctrl Pts',(17.4307631168861,-20.6203162675398,-11.5755106941243));
#83655=CARTESIAN_POINT('Ctrl Pts',(17.4339824273816,-20.622821148724,-11.5752642839514));
#83656=CARTESIAN_POINT('Ctrl Pts',(17.4339917617322,-20.6228284114701,-11.5752635694872));
#83657=CARTESIAN_POINT('Ctrl Pts',(17.4340104667637,-20.6228429649781,-11.5752621377762));
#83658=CARTESIAN_POINT('Ctrl Pts',(17.4340198369046,-20.622850255319,-11.5752614205706));
#83659=CARTESIAN_POINT('Ctrl Pts',(17.434038613452,-20.622864863963,-11.5752599833818));
#83660=CARTESIAN_POINT('Ctrl Pts',(17.4340480202258,-20.6228721825511,-11.5752592633703));
#83661=CARTESIAN_POINT('Ctrl Pts',(17.43406687066,-20.62288684817,-11.5752578205222));
#83662=CARTESIAN_POINT('Ctrl Pts',(17.4340763137596,-20.6228941947635,-11.5752570977284));
#83663=CARTESIAN_POINT('Ctrl Pts',(17.4340959153776,-20.6229094442691,-11.5752555973791));
#83664=CARTESIAN_POINT('Ctrl Pts',(17.4341060746042,-20.622917347712,-11.5752548197693));
#83665=CARTESIAN_POINT('Ctrl Pts',(17.4341265700933,-20.622933292024,-11.5752532509966));
#83666=CARTESIAN_POINT('Ctrl Pts',(17.4341369060107,-20.6229413326195,-11.5752524598602));
#83667=CARTESIAN_POINT('Ctrl Pts',(17.4341577587443,-20.622957554226,-11.5752508637384));
#83668=CARTESIAN_POINT('Ctrl Pts',(17.4341682755815,-20.6229657352479,-11.5752500587515));
#83669=CARTESIAN_POINT('Ctrl Pts',(17.4341894938998,-20.6229822406045,-11.5752484346421));
#83670=CARTESIAN_POINT('Ctrl Pts',(17.4342001953889,-20.6229905649394,-11.5752476155189));
#83671=CARTESIAN_POINT('Ctrl Pts',(17.4342217871971,-20.6230073601613,-11.5752459628165));
#83672=CARTESIAN_POINT('Ctrl Pts',(17.4342326771934,-20.6230158307911,-11.5752451292618));
#83673=CARTESIAN_POINT('Ctrl Pts',(17.434254650104,-20.6230329217645,-11.5752434473833));
#83674=CARTESIAN_POINT('Ctrl Pts',(17.434265732831,-20.6230415419563,-11.5752425990738));
#83675=CARTESIAN_POINT('Ctrl Pts',(17.4342880948555,-20.6230589348763,-11.5752408874057));
#83676=CARTESIAN_POINT('Ctrl Pts',(17.4342993746865,-20.623067708013,-11.5752400240064));
#83677=CARTESIAN_POINT('Ctrl Pts',(17.4343221353084,-20.6230854102177,-11.5752382818227));
#83678=CARTESIAN_POINT('Ctrl Pts',(17.4343336161257,-20.6230943392994,-11.5752374030362));
#83679=CARTESIAN_POINT('Ctrl Pts',(17.4343567834148,-20.6231123570255,-11.5752356297187));
#83680=CARTESIAN_POINT('Ctrl Pts',(17.4343684697384,-20.6231214455476,-11.575234735199));
#83681=CARTESIAN_POINT('Ctrl Pts',(17.4343920522796,-20.6231397854306,-11.5752329300904));
#83682=CARTESIAN_POINT('Ctrl Pts',(17.4344039488733,-20.6231490370769,-11.5752320194727));
#83683=CARTESIAN_POINT('Ctrl Pts',(17.4344279569348,-20.6231677070596,-11.5752301817866));
#83684=CARTESIAN_POINT('Ctrl Pts',(17.4344400680302,-20.6231771250989,-11.5752292547467));
#83685=CARTESIAN_POINT('Ctrl Pts',(17.4344645098804,-20.6231961315667,-11.5752273838499));
#83686=CARTESIAN_POINT('Ctrl Pts',(17.4344768406379,-20.6232057199895,-11.5752264399927));
#83687=CARTESIAN_POINT('Ctrl Pts',(17.4345017265397,-20.6232250708766,-11.5752245350993));
#83688=CARTESIAN_POINT('Ctrl Pts',(17.4345142817885,-20.6232348334143,-11.5752235740549));
#83689=CARTESIAN_POINT('Ctrl Pts',(17.4345396217877,-20.623254536484,-11.5752216343955));
#83690=CARTESIAN_POINT('Ctrl Pts',(17.4345524065069,-20.6232644769836,-11.5752206557827));
#83691=CARTESIAN_POINT('Ctrl Pts',(17.4372579127235,-20.6253680387425,-11.5750135610604));
#83692=CARTESIAN_POINT('Ctrl Pts',(17.4399556321339,-20.6274551045601,-11.5748069784263));
#83693=CARTESIAN_POINT('Ctrl Pts',(17.4462816455741,-20.6323247742902,-11.5743223663908));
#83694=CARTESIAN_POINT('Ctrl Pts',(17.4499139066277,-20.6351021393012,-11.5740439728026));
#83695=CARTESIAN_POINT('Ctrl Pts',(17.4610839464052,-20.643585972655,-11.5731874952056));
#83696=CARTESIAN_POINT('Ctrl Pts',(17.4686508572441,-20.6492536409409,-11.5726068015111));
#83697=CARTESIAN_POINT('Ctrl Pts',(17.5750299268252,-20.7278255136771,-11.5644392897217));
#83698=CARTESIAN_POINT('Ctrl Pts',(17.6799538290228,-20.7920401182624,-11.5563501677246));
#83699=CARTESIAN_POINT('Ctrl Pts',(17.8839337949351,-20.8936821142843,-11.5412917490764));
#83700=CARTESIAN_POINT('Ctrl Pts',(17.9814010562225,-20.9334994232368,-11.534347998024));
#83701=CARTESIAN_POINT('Ctrl Pts',(18.1338418360431,-20.9828950547948,-11.5240479729228));
#83702=CARTESIAN_POINT('Ctrl Pts',(18.1869009012604,-20.9978269580655,-11.520559119859));
#83703=CARTESIAN_POINT('Ctrl Pts',(18.2738420581457,-21.0186688752732,-11.5150019494289));
#83704=CARTESIAN_POINT('Ctrl Pts',(18.3073890142597,-21.0258536241991,-11.5128952001977));
#83705=CARTESIAN_POINT('Ctrl Pts',(18.3517178012349,-21.0342262456084,-11.5101587984258));
#83706=CARTESIAN_POINT('Ctrl Pts',(18.3623535907935,-21.0361508512346,-11.5095058072679));
#83707=CARTESIAN_POINT('Ctrl Pts',(18.3798007419064,-21.0391702056683,-11.5084403237669));
#83708=CARTESIAN_POINT('Ctrl Pts',(18.3866034436415,-21.0403132466768,-11.5080263020698));
#83709=CARTESIAN_POINT('Ctrl Pts',(18.3997843219157,-21.0424618078854,-11.507226788781));
#83710=CARTESIAN_POINT('Ctrl Pts',(18.4061617425628,-21.0434714361165,-11.5068411708662));
#83711=CARTESIAN_POINT('Ctrl Pts',(18.4209004478961,-21.0457356932661,-11.5059527427402));
#83712=CARTESIAN_POINT('Ctrl Pts',(18.4292648647372,-21.0469694468616,-11.5054505986319));
#83713=CARTESIAN_POINT('Ctrl Pts',(18.4517859894326,-21.0501535837854,-11.5041039590927));
#83714=CARTESIAN_POINT('Ctrl Pts',(18.4659555796157,-21.0520108124781,-11.5032624052741));
#83715=CARTESIAN_POINT('Ctrl Pts',(18.5961652861964,-21.0677381954921,-11.4955788498022));
#83716=CARTESIAN_POINT('Ctrl Pts',(18.7131556084473,-21.0721220006379,-11.4890537017563));
#83717=CARTESIAN_POINT('Ctrl Pts',(18.9926300454236,-21.0594457029593,-11.4737384312352));
#83718=CARTESIAN_POINT('Ctrl Pts',(19.1539211072279,-21.0333147873812,-11.4651317675645));
#83719=CARTESIAN_POINT('Ctrl Pts',(19.3417341561108,-20.9801506513749,-11.4539222201374));
#83720=CARTESIAN_POINT('Ctrl Pts',(19.372658243819,-20.9706260820052,-11.4520348788544));
#83721=CARTESIAN_POINT('Ctrl Pts',(19.4102082543697,-20.9581115764149,-11.4496781635906));
#83722=CARTESIAN_POINT('Ctrl Pts',(19.4170546614957,-20.9557908040222,-11.4492457962696));
#83723=CARTESIAN_POINT('Ctrl Pts',(19.4277721090722,-20.9520965305072,-11.4485645678286));
#83724=CARTESIAN_POINT('Ctrl Pts',(19.4316513414119,-20.9507467262863,-11.4483170873816));
#83725=CARTESIAN_POINT('Ctrl Pts',(19.4388970201079,-20.948201881626,-11.4478531006819));
#83726=CARTESIAN_POINT('Ctrl Pts',(19.4422643782183,-20.9470096067571,-11.4476367589405));
#83727=CARTESIAN_POINT('Ctrl Pts',(19.4499468844092,-20.944267572622,-11.4471415728569));
#83728=CARTESIAN_POINT('Ctrl Pts',(19.4542600107789,-20.9427123192907,-11.4468624054466));
#83729=CARTESIAN_POINT('Ctrl Pts',(19.4675111947637,-20.9378854247326,-11.4460012274905));
#83730=CARTESIAN_POINT('Ctrl Pts',(19.476432123959,-20.9345675591387,-11.4454165662993));
#83731=CARTESIAN_POINT('Ctrl Pts',(19.5577862152014,-20.9036843226468,-11.4400418365533));
#83732=CARTESIAN_POINT('Ctrl Pts',(19.6286695134842,-20.8722237390315,-11.4350484837293));
#83733=CARTESIAN_POINT('Ctrl Pts',(19.73407924571,-20.8183342422861,-11.4273007178977));
#83734=CARTESIAN_POINT('Ctrl Pts',(19.7699503063158,-20.798664245764,-11.4246034109206));
#83735=CARTESIAN_POINT('Ctrl Pts',(19.8995680070527,-20.7226223033766,-11.4146765282574));
#83736=CARTESIAN_POINT('Ctrl Pts',(19.9894839907786,-20.6600443598228,-11.4074442175789));
#83737=CARTESIAN_POINT('Ctrl Pts',(20.1168138872927,-20.5559170891765,-11.3968715951581));
#83738=CARTESIAN_POINT('Ctrl Pts',(20.1580871526203,-20.5193866397022,-11.3933829028324));
#83739=CARTESIAN_POINT('Ctrl Pts',(20.2226688194853,-20.4575665516544,-11.3878259584399));
#83740=CARTESIAN_POINT('Ctrl Pts',(20.2468675784327,-20.433248595597,-11.3857192784057));
#83741=CARTESIAN_POINT('Ctrl Pts',(20.2779010987559,-20.400507926076,-11.3829829519992));
#83742=CARTESIAN_POINT('Ctrl Pts',(20.2852762497047,-20.3926067536049,-11.3823299686178));
#83743=CARTESIAN_POINT('Ctrl Pts',(20.2972587535368,-20.3795708917489,-11.3812644945531));
#83744=CARTESIAN_POINT('Ctrl Pts',(20.3019020239034,-20.3744696224067,-11.3808504745681));
#83745=CARTESIAN_POINT('Ctrl Pts',(20.3108431706396,-20.3645495761415,-11.380050962339));
#83746=CARTESIAN_POINT('Ctrl Pts',(20.3151440917833,-20.3597336581523,-11.3796653437835));
#83747=CARTESIAN_POINT('Ctrl Pts',(20.3250258065048,-20.3485662773322,-11.3787769109711));
#83748=CARTESIAN_POINT('Ctrl Pts',(20.3305907420744,-20.3422008809634,-11.3782747628394));
#83749=CARTESIAN_POINT('Ctrl Pts',(20.3454585502765,-20.3249874567626,-11.3769281053858));
#83750=CARTESIAN_POINT('Ctrl Pts',(20.3546900645286,-20.3140781715222,-11.3760865377999));
#83751=CARTESIAN_POINT('Ctrl Pts',(20.4384059652236,-20.2130912128594,-11.3684019128798));
#83752=CARTESIAN_POINT('Ctrl Pts',(20.5054258000469,-20.1170779562622,-11.3618758147859));
#83753=CARTESIAN_POINT('Ctrl Pts',(20.6460722948785,-19.8751547911064,-11.3465565665481));
#83754=CARTESIAN_POINT('Ctrl Pts',(20.7114169631579,-19.7253339817636,-11.3379470373315));
#83755=CARTESIAN_POINT('Ctrl Pts',(20.7683513185978,-19.5386398338669,-11.3267372466973));
#83756=CARTESIAN_POINT('Ctrl Pts',(20.7770615655289,-19.5075454664342,-11.3248536759389));
#83757=CARTESIAN_POINT('Ctrl Pts',(20.7868459593231,-19.4692665286364,-11.322501156041));
#83758=CARTESIAN_POINT('Ctrl Pts',(20.7885992210691,-19.4622580050491,-11.3220690583001));
#83759=CARTESIAN_POINT('Ctrl Pts',(20.7912926926222,-19.4512520799288,-11.3213881610939));
#83760=CARTESIAN_POINT('Ctrl Pts',(20.7922572222017,-19.4472606071817,-11.3211407400853));
#83761=CARTESIAN_POINT('Ctrl Pts',(20.7940391320323,-19.4397914889639,-11.3206768035368));
#83762=CARTESIAN_POINT('Ctrl Pts',(20.7948593248133,-19.4363145722366,-11.320460452135));
#83763=CARTESIAN_POINT('Ctrl Pts',(20.7967124502302,-19.4283689576754,-11.3199651629888));
#83764=CARTESIAN_POINT('Ctrl Pts',(20.7977396600296,-19.4238989837647,-11.3196859016558));
#83765=CARTESIAN_POINT('Ctrl Pts',(20.8008555854555,-19.4101350561564,-11.3188241522013));
#83766=CARTESIAN_POINT('Ctrl Pts',(20.8028960697313,-19.40083046428,-11.3182390084326));
#83767=CARTESIAN_POINT('Ctrl Pts',(20.8297138336639,-19.274471861711,-11.3102604968273));
#83768=CARTESIAN_POINT('Ctrl Pts',(20.8445842122161,-19.155549064988,-11.3023899189407));
#83769=CARTESIAN_POINT('Ctrl Pts',(20.8564950518746,-18.8556874059274,-11.2825645407231));
#83770=CARTESIAN_POINT('Ctrl Pts',(20.8405691200868,-18.6751359406159,-11.2707105169302));
#83771=CARTESIAN_POINT('Ctrl Pts',(20.7973522962586,-18.4779529803882,-11.2583119260309));
#83772=CARTESIAN_POINT('Ctrl Pts',(20.7924749720833,-18.4572029540042,-11.2570128401839));
#83773=CARTESIAN_POINT('Ctrl Pts',(20.7850943720238,-18.427803647045,-11.255179722248));
#83774=CARTESIAN_POINT('Ctrl Pts',(20.7828481455969,-18.4190917343587,-11.2546374496952));
#83775=CARTESIAN_POINT('Ctrl Pts',(20.7788773590873,-18.4040874629557,-11.2537050522803));
#83776=CARTESIAN_POINT('Ctrl Pts',(20.7771791354058,-18.397788321957,-11.2533140810688));
#83777=CARTESIAN_POINT('Ctrl Pts',(20.7738718502158,-18.3857425983033,-11.2525673006876));
#83778=CARTESIAN_POINT('Ctrl Pts',(20.772267558791,-18.3799947813332,-11.2522113409767));
#83779=CARTESIAN_POINT('Ctrl Pts',(20.7680328005942,-18.3650666463349,-11.2512877930991));
#83780=CARTESIAN_POINT('Ctrl Pts',(20.7653644631293,-18.3558971414135,-11.2507214421635));
#83781=CARTESIAN_POINT('Ctrl Pts',(20.7560548436776,-18.3246940293383,-11.2487971282787));
#83782=CARTESIAN_POINT('Ctrl Pts',(20.7491162434409,-18.3027503113763,-11.2474488748676));
#83783=CARTESIAN_POINT('Ctrl Pts',(20.6862858652122,-18.1147655702311,-11.2359316270504));
#83784=CARTESIAN_POINT('Ctrl Pts',(20.610342576037,-17.9561451711754,-11.226510631122));
#83785=CARTESIAN_POINT('Ctrl Pts',(20.4686207712067,-17.7352895460093,-11.212232970457));
#83786=CARTESIAN_POINT('Ctrl Pts',(20.4170386329782,-17.6648822502407,-11.2074595508535));
#83787=CARTESIAN_POINT('Ctrl Pts',(20.3370414771626,-17.5687496806177,-11.2003194528138));
#83788=CARTESIAN_POINT('Ctrl Pts',(20.3120403183255,-17.5402947274221,-11.1981195543073));
#83789=CARTESIAN_POINT('Ctrl Pts',(20.2811408986288,-17.5069735593155,-11.1954158292783));
#83790=CARTESIAN_POINT('Ctrl Pts',(20.2759608043423,-17.5014472610656,-11.1949630568863));
#83791=CARTESIAN_POINT('Ctrl Pts',(20.2678743007375,-17.4929125707651,-11.1942567783261));
#83792=CARTESIAN_POINT('Ctrl Pts',(20.2649883835013,-17.4898847290643,-11.1940048250653));
#83793=CARTESIAN_POINT('Ctrl Pts',(20.2596271493294,-17.4842931146069,-11.1935369125596));
#83794=CARTESIAN_POINT('Ctrl Pts',(20.2571543251906,-17.4817270317136,-11.1933211454175));
#83795=CARTESIAN_POINT('Ctrl Pts',(20.2515587020548,-17.4759496451661,-11.1928330220693));
#83796=CARTESIAN_POINT('Ctrl Pts',(20.2484322014706,-17.4727420203078,-11.1925603790894));
#83797=CARTESIAN_POINT('Ctrl Pts',(20.2392018825856,-17.4633321331643,-11.1917557943067));
#83798=CARTESIAN_POINT('Ctrl Pts',(20.2330700610129,-17.4571576433272,-11.1912217263059));
#83799=CARTESIAN_POINT('Ctrl Pts',(20.1893037431093,-17.4136268759787,-11.1874139730482));
#83800=CARTESIAN_POINT('Ctrl Pts',(20.150318558489,-17.3776615438736,-11.184044363763));
#83801=CARTESIAN_POINT('Ctrl Pts',(20.0956697262834,-17.330919632673,-11.1793977600611));
#83802=CARTESIAN_POINT('Ctrl Pts',(20.0811475307665,-17.3188314534767,-11.1781699099195));
#83803=CARTESIAN_POINT('Ctrl Pts',(19.9523449682026,-17.2145039755766,-11.1673523549762));
#83804=CARTESIAN_POINT('Ctrl Pts',(19.8289029615913,-17.134185476818,-11.1575172365772));
#83805=CARTESIAN_POINT('Ctrl Pts',(19.6432086155032,-17.0391915892997,-11.1440421205149));
#83806=CARTESIAN_POINT('Ctrl Pts',(19.5870697377721,-17.0135032962788,-11.1401175683879));
#83807=CARTESIAN_POINT('Ctrl Pts',(19.4954010172047,-16.9763121910109,-11.1339536533744));
#83808=CARTESIAN_POINT('Ctrl Pts',(19.4605532315251,-16.9632329183491,-11.1316645689448));
#83809=CARTESIAN_POINT('Ctrl Pts',(19.4148571025361,-16.9474435690025,-11.128730560912));
#83810=CARTESIAN_POINT('Ctrl Pts',(19.4043086281309,-16.943891629022,-11.1280578773836));
#83811=CARTESIAN_POINT('Ctrl Pts',(19.3871106333284,-16.9382512406276,-11.1269684872809));
#83812=CARTESIAN_POINT('Ctrl Pts',(19.3804780510407,-16.9361121815512,-11.1265501168865));
#83813=CARTESIAN_POINT('Ctrl Pts',(19.3677046436966,-16.9320621832838,-11.1257477388487));
#83814=CARTESIAN_POINT('Ctrl Pts',(19.3615654459575,-16.9301464021121,-11.1253635757175));
#83815=CARTESIAN_POINT('Ctrl Pts',(19.3474914930732,-16.9258248017762,-11.1244862267832));
#83816=CARTESIAN_POINT('Ctrl Pts',(19.3395511111717,-16.9234375531636,-11.123993653672));
#83817=CARTESIAN_POINT('Ctrl Pts',(19.3184249267719,-16.9172211358404,-11.1226894014822));
#83818=CARTESIAN_POINT('Ctrl Pts',(19.3052154127258,-16.9134734520792,-11.1218803780707));
#83819=CARTESIAN_POINT('Ctrl Pts',(19.204594536313,-16.8859810703903,-11.1157650702585));
#83820=CARTESIAN_POINT('Ctrl Pts',(19.1157711315264,-16.8677382295575,-11.1106426004892));
#83821=CARTESIAN_POINT('Ctrl Pts',(18.8872940776131,-16.8359152511998,-11.0978743564297));
#83822=CARTESIAN_POINT('Ctrl Pts',(18.7469761208272,-16.8304101750477,-11.0904248980446));
#83823=CARTESIAN_POINT('Ctrl Pts',(18.5526132765211,-16.8420776196516,-11.0796641828763));
#83824=CARTESIAN_POINT('Ctrl Pts',(18.4982307953527,-16.8474607033818,-11.0766013706266));
#83825=CARTESIAN_POINT('Ctrl Pts',(18.4161300202232,-16.8588095725219,-11.0718193560586));
#83826=CARTESIAN_POINT('Ctrl Pts',(18.3882204273055,-16.8632386922141,-11.070165651825));
#83827=CARTESIAN_POINT('Ctrl Pts',(18.3535925120223,-16.8694469737997,-11.0680695012531));
#83828=CARTESIAN_POINT('Ctrl Pts',(18.3467817566077,-16.8707025698366,-11.0676550730619));
#83829=CARTESIAN_POINT('Ctrl Pts',(18.3360076676299,-16.8727435397262,-11.0669958992063));
#83830=CARTESIAN_POINT('Ctrl Pts',(18.332040141934,-16.8735068929412,-11.0667523900545));
#83831=CARTESIAN_POINT('Ctrl Pts',(18.3245570934836,-16.8749688607651,-11.0662916177653));
#83832=CARTESIAN_POINT('Ctrl Pts',(18.3210411510002,-16.8756650474065,-11.0660744937299));
#83833=CARTESIAN_POINT('Ctrl Pts',(18.3130009792761,-16.8772782995604,-11.0655765552337));
#83834=CARTESIAN_POINT('Ctrl Pts',(18.308477975333,-16.8782012355781,-11.0652954091011));
#83835=CARTESIAN_POINT('Ctrl Pts',(18.2964661197226,-16.880693250898,-11.0645460883637));
#83836=CARTESIAN_POINT('Ctrl Pts',(18.2889827743871,-16.8822881335517,-11.0640764979191));
#83837=CARTESIAN_POINT('Ctrl Pts',(18.2362947215605,-16.8938161902402,-11.0607515242731));
#83838=CARTESIAN_POINT('Ctrl Pts',(18.191421248772,-16.9051881548201,-11.0578225841764));
#83839=CARTESIAN_POINT('Ctrl Pts',(18.14178032646,-16.919515331774,-11.0544997195492));
#83840=CARTESIAN_POINT('Ctrl Pts',(18.1366060246779,-16.921030156378,-11.054152343825));
#83841=CARTESIAN_POINT('Ctrl Pts',(18.1271058068358,-16.9238508790084,-11.053512739365));
#83842=CARTESIAN_POINT('Ctrl Pts',(18.1227781631577,-16.9251508974827,-11.0532206875028));
#83843=CARTESIAN_POINT('Ctrl Pts',(18.0946975268686,-16.9336843962723,-11.0513212923962));
#83844=CARTESIAN_POINT('Ctrl Pts',(18.0710697440528,-16.9413212731072,-11.0497027884841));
#83845=CARTESIAN_POINT('Ctrl Pts',(18.0104644642029,-16.9620942411824,-11.0455069299301));
#83846=CARTESIAN_POINT('Ctrl Pts',(17.9737080802997,-16.9758459856872,-11.0429190771497));
#83847=CARTESIAN_POINT('Ctrl Pts',(17.8360959793658,-17.0317389663027,-11.0331074211231));
#83848=CARTESIAN_POINT('Ctrl Pts',(17.7381652476012,-17.0806500375686,-11.02588107901));
#83849=CARTESIAN_POINT('Ctrl Pts',(17.5972933601307,-17.1652119986825,-11.015320990367));
#83850=CARTESIAN_POINT('Ctrl Pts',(17.5512599991049,-17.1953440138584,-11.0118388218654));
#83851=CARTESIAN_POINT('Ctrl Pts',(17.4785407929527,-17.2470998284689,-11.0062910529837));
#83852=CARTESIAN_POINT('Ctrl Pts',(17.4511174492235,-17.2676381054598,-11.0041871826606));
#83853=CARTESIAN_POINT('Ctrl Pts',(17.4157162757556,-17.2955176652298,-11.0014539166859));
#83854=CARTESIAN_POINT('Ctrl Pts',(17.4072804090453,-17.3022664346126,-11.0008012492629));
#83855=CARTESIAN_POINT('Ctrl Pts',(17.3935441124593,-17.3134291045566,-10.999736158596));
#83856=CARTESIAN_POINT('Ctrl Pts',(17.3882130164572,-17.3178047966921,-10.9993222081741));
#83857=CARTESIAN_POINT('Ctrl Pts',(17.377932189508,-17.3263275886207,-10.9985227389518));
#83858=CARTESIAN_POINT('Ctrl Pts',(17.372979868802,-17.3304714311267,-10.9981370943185));
#83859=CARTESIAN_POINT('Ctrl Pts',(17.3615850302572,-17.3400950145774,-10.9972484708676));
#83860=CARTESIAN_POINT('Ctrl Pts',(17.3551562084127,-17.3455908576044,-10.996746159093));
#83861=CARTESIAN_POINT('Ctrl Pts',(17.3379467303153,-17.3604822465446,-10.9953987729137));
#83862=CARTESIAN_POINT('Ctrl Pts',(17.3272279335409,-17.369948844274,-10.9945566452876));
#83863=CARTESIAN_POINT('Ctrl Pts',(17.2292160340306,-17.4582945268088,-10.9868265710336));
#83864=CARTESIAN_POINT('Ctrl Pts',(17.1485393408821,-17.5442178203698,-10.980260094241));
#83865=CARTESIAN_POINT('Ctrl Pts',(16.9737389814325,-17.7645919269791,-10.964865573814));
#83866=CARTESIAN_POINT('Ctrl Pts',(16.8872806441647,-17.9041106665782,-10.9562204796831));
#83867=CARTESIAN_POINT('Ctrl Pts',(16.8045807838236,-18.0802252941688,-10.9450299580342));
#83868=CARTESIAN_POINT('Ctrl Pts',(16.7920251371487,-18.1085647309433,-10.9432200679027));
#83869=CARTESIAN_POINT('Ctrl Pts',(16.7773512455334,-18.1437515631972,-10.9409495882056));
#83870=CARTESIAN_POINT('Ctrl Pts',(16.7746389808509,-18.1503490302559,-10.9405228834263));
#83871=CARTESIAN_POINT('Ctrl Pts',(16.7704255502637,-18.1607471465774,-10.9398486139372));
#83872=CARTESIAN_POINT('Ctrl Pts',(16.7689019287588,-18.1645387200241,-10.9396023836658));
#83873=CARTESIAN_POINT('Ctrl Pts',(16.7660657187922,-18.1716561979109,-10.9391394394251));
#83874=CARTESIAN_POINT('Ctrl Pts',(16.7647505755518,-18.1749810245281,-10.9389228820742));
#83875=CARTESIAN_POINT('Ctrl Pts',(16.7617562476082,-18.1826074444657,-10.9384254716461));
#83876=CARTESIAN_POINT('Ctrl Pts',(16.7600827149832,-18.1869111983962,-10.9381442843083));
#83877=CARTESIAN_POINT('Ctrl Pts',(16.7549425689768,-18.2002590221147,-10.9372707676825));
#83878=CARTESIAN_POINT('Ctrl Pts',(16.751523990189,-18.2093212838226,-10.9366756787059));
#83879=CARTESIAN_POINT('Ctrl Pts',(16.7114754927785,-18.3177322694258,-10.9295352455752));
#83880=CARTESIAN_POINT('Ctrl Pts',(16.682291093586,-18.41965971884,-10.9226144770236));
#83881=CARTESIAN_POINT('Ctrl Pts',(16.631792491142,-18.6638812142766,-10.906164778877));
#83882=CARTESIAN_POINT('Ctrl Pts',(16.6170952312567,-18.8070440704221,-10.8966461771693));
#83883=CARTESIAN_POINT('Ctrl Pts',(16.6169595357191,-19.0125966091521,-10.8835935545742));
#83884=CARTESIAN_POINT('Ctrl Pts',(16.6196417426175,-19.0745670565041,-10.8797325121679));
#83885=CARTESIAN_POINT('Ctrl Pts',(16.6261219965063,-19.1487067147389,-10.8751997242484));
#83886=CARTESIAN_POINT('Ctrl Pts',(16.6273121374462,-19.1610680973189,-10.8744468127296));
#83887=CARTESIAN_POINT('Ctrl Pts',(16.6294460867429,-19.1813590546165,-10.8732154416387));
#83888=CARTESIAN_POINT('Ctrl Pts',(16.6303260989716,-19.1892949021742,-10.8727349862853));
#83889=CARTESIAN_POINT('Ctrl Pts',(16.6319896970467,-19.2035598412311,-10.8718733420666));
#83890=CARTESIAN_POINT('Ctrl Pts',(16.6327570210474,-19.2098906982097,-10.8714916456779));
#83891=CARTESIAN_POINT('Ctrl Pts',(16.6344530082202,-19.2233732415897,-10.870680230157));
#83892=CARTESIAN_POINT('Ctrl Pts',(16.6353896338161,-19.2305238586969,-10.8702507673755));
#83893=CARTESIAN_POINT('Ctrl Pts',(16.6380125543551,-19.2497836446978,-10.8690963293766));
#83894=CARTESIAN_POINT('Ctrl Pts',(16.6397672532445,-19.261883338077,-10.8683735208393));
#83895=CARTESIAN_POINT('Ctrl Pts',(16.6490971357875,-19.3225155647284,-10.8647629875313));
#83896=CARTESIAN_POINT('Ctrl Pts',(16.6582553255207,-19.3707915175288,-10.8619257816648));
#83897=CARTESIAN_POINT('Ctrl Pts',(16.688975743057,-19.5067116773627,-10.8540036597052));
#83898=CARTESIAN_POINT('Ctrl Pts',(16.7144720710822,-19.5933556444856,-10.8490363862048));
#83899=CARTESIAN_POINT('Ctrl Pts',(16.7454194496957,-19.67811045644,-10.8441190240937));
#83900=CARTESIAN_POINT('Origin',(18.734,-18.952,0.));
#83901=CARTESIAN_POINT('',(16.7454194499602,-19.6781104571642,-10.0464611570501));
#83902=CARTESIAN_POINT('',(16.7460269997162,-19.677879090888,-10.2662522551303));
#83903=CARTESIAN_POINT('',(16.7454194499637,-19.6781104571739,0.));
#83904=CARTESIAN_POINT('',(16.614176999282,-18.9530774369803,-10.3109437209775));
#83905=CARTESIAN_POINT('Ctrl Pts',(16.7460269997163,-19.6778790908883,-10.2662522551303));
#83906=CARTESIAN_POINT('Ctrl Pts',(16.6804601656347,-19.5036328070715,-10.2774434318562));
#83907=CARTESIAN_POINT('Ctrl Pts',(16.6235838006535,-19.2611105659415,-10.2923405871386));
#83908=CARTESIAN_POINT('Ctrl Pts',(16.6137958948767,-19.0144660751781,-10.307237742421));
#83909=CARTESIAN_POINT('Ctrl Pts',(16.614176999282,-18.9530774369803,-10.3109437209775));
#83910=CARTESIAN_POINT('Ctrl Pts',(16.6170002227488,-18.9529711427249,-10.3093226184743));
#83911=CARTESIAN_POINT('Ctrl Pts',(16.616920601068,-18.7794033692573,-10.3204871727274));
#83912=CARTESIAN_POINT('Ctrl Pts',(16.6381853782203,-18.6064738253141,-10.3321971334834));
#83913=CARTESIAN_POINT('Ctrl Pts',(16.6951945281285,-18.3786675872106,-10.347362818657));
#83914=CARTESIAN_POINT('Ctrl Pts',(16.7126292170894,-18.3199406142348,-10.3512558888495));
#83915=CARTESIAN_POINT('Ctrl Pts',(16.7446483001179,-18.2270596950899,-10.3573763525111));
#83916=CARTESIAN_POINT('Ctrl Pts',(16.7576257037044,-18.1923925068387,-10.3596526032797));
#83917=CARTESIAN_POINT('Ctrl Pts',(16.7756718658497,-18.1477840385356,-10.3625727652533));
#83918=CARTESIAN_POINT('Ctrl Pts',(16.7799187407749,-18.1375192860528,-10.3632441131218));
#83919=CARTESIAN_POINT('Ctrl Pts',(16.7869592378109,-18.1208743967158,-10.364331881253));
#83920=CARTESIAN_POINT('Ctrl Pts',(16.7897038552785,-18.114473880118,-10.3647499560836));
#83921=CARTESIAN_POINT('Ctrl Pts',(16.795044322094,-18.1021875158721,-10.3655521292429));
#83922=CARTESIAN_POINT('Ctrl Pts',(16.7976355092999,-18.0962997372738,-10.3659363811201));
#83923=CARTESIAN_POINT('Ctrl Pts',(16.803632170112,-18.0828406585491,-10.3668144346507));
#83924=CARTESIAN_POINT('Ctrl Pts',(16.8070554379508,-18.0752773658198,-10.3673076202088));
#83925=CARTESIAN_POINT('Ctrl Pts',(16.8162731215175,-18.0552268295972,-10.3686145711229));
#83926=CARTESIAN_POINT('Ctrl Pts',(16.8221450549382,-18.0427755051673,-10.3694256630356));
#83927=CARTESIAN_POINT('Ctrl Pts',(16.86816945609,-17.9475992362546,-10.3756234047571));
#83928=CARTESIAN_POINT('Ctrl Pts',(16.9135543444935,-17.8675069712912,-10.3808202622217));
#83929=CARTESIAN_POINT('Ctrl Pts',(17.0412308323666,-17.6729240859934,-10.3936931494177));
#83930=CARTESIAN_POINT('Ctrl Pts',(17.129993379071,-17.5632368212038,-10.4011754664971));
#83931=CARTESIAN_POINT('Ctrl Pts',(17.2663405273322,-17.4254068468746,-10.4119025284124));
#83932=CARTESIAN_POINT('Ctrl Pts',(17.3051057925353,-17.3890631632552,-10.414884573204));
#83933=CARTESIAN_POINT('Ctrl Pts',(17.3590975317378,-17.3421330583069,-10.4190145946725));
#83934=CARTESIAN_POINT('Ctrl Pts',(17.3731579458471,-17.3302302185466,-10.4200881377047));
#83935=CARTESIAN_POINT('Ctrl Pts',(17.3941500956425,-17.3129245248535,-10.4216910836558));
#83936=CARTESIAN_POINT('Ctrl Pts',(17.4009633778602,-17.3073786035323,-10.4222113642647));
#83937=CARTESIAN_POINT('Ctrl Pts',(17.4132981893964,-17.2974652353411,-10.4231537311002));
#83938=CARTESIAN_POINT('Ctrl Pts',(17.4188074014079,-17.2930825863118,-10.4235747878974));
#83939=CARTESIAN_POINT('Ctrl Pts',(17.4275362937868,-17.2862094511804,-10.4242423503102));
#83940=CARTESIAN_POINT('Ctrl Pts',(17.4307415303657,-17.2837005877618,-10.4244875695442));
#83941=CARTESIAN_POINT('Ctrl Pts',(17.4339632609263,-17.2811937643168,-10.4247341645007));
#83942=CARTESIAN_POINT('Ctrl Pts',(17.4339725707876,-17.2811865204534,-10.4247348770892));
#83943=CARTESIAN_POINT('Ctrl Pts',(17.4339912262073,-17.2811720052016,-10.4247363050002));
#83944=CARTESIAN_POINT('Ctrl Pts',(17.434000571806,-17.2811647337827,-10.4247370203259));
#83945=CARTESIAN_POINT('Ctrl Pts',(17.434019299241,-17.2811501630023,-10.424738453753));
#83946=CARTESIAN_POINT('Ctrl Pts',(17.4340286808851,-17.2811428637912,-10.4247391718396));
#83947=CARTESIAN_POINT('Ctrl Pts',(17.4340474803129,-17.2811282375055,-10.424740610781));
#83948=CARTESIAN_POINT('Ctrl Pts',(17.4340568986222,-17.2811209100229,-10.424741331676));
#83949=CARTESIAN_POINT('Ctrl Pts',(17.4340757716204,-17.2811062270105,-10.4247427762524));
#83950=CARTESIAN_POINT('Ctrl Pts',(17.4340852265746,-17.2810988712752,-10.4247434999543));
#83951=CARTESIAN_POINT('Ctrl Pts',(17.4341048926039,-17.281083571828,-10.424745005235));
#83952=CARTESIAN_POINT('Ctrl Pts',(17.434115103232,-17.2810756284853,-10.4247457867799));
#83953=CARTESIAN_POINT('Ctrl Pts',(17.4341357027151,-17.2810596034516,-10.4247473635138));
#83954=CARTESIAN_POINT('Ctrl Pts',(17.4341460916624,-17.2810515216941,-10.42474815871));
#83955=CARTESIAN_POINT('Ctrl Pts',(17.4341670515367,-17.2810352169275,-10.424749763034));
#83956=CARTESIAN_POINT('Ctrl Pts',(17.4341776223344,-17.2810269940244,-10.4247505721519));
#83957=CARTESIAN_POINT('Ctrl Pts',(17.4341989499914,-17.2810104038079,-10.4247522046319));
#83958=CARTESIAN_POINT('Ctrl Pts',(17.4342097065417,-17.2810020367405,-10.4247530279704));
#83959=CARTESIAN_POINT('Ctrl Pts',(17.4342314092451,-17.2809851554581,-10.4247546891626));
#83960=CARTESIAN_POINT('Ctrl Pts',(17.4342423558561,-17.2809766408928,-10.4247555270515));
#83961=CARTESIAN_POINT('Ctrl Pts',(17.4342644429403,-17.2809594613194,-10.4247572176708));
#83962=CARTESIAN_POINT('Ctrl Pts',(17.4342755832488,-17.2809507964456,-10.4247580703887));
#83963=CARTESIAN_POINT('Ctrl Pts',(17.4342980620022,-17.2809333129492,-10.4247597909932));
#83964=CARTESIAN_POINT('Ctrl Pts',(17.4343094004992,-17.2809244942925,-10.4247606588839));
#83965=CARTESIAN_POINT('Ctrl Pts',(17.4343322799526,-17.2809066998876,-10.4247624101651));
#83966=CARTESIAN_POINT('Ctrl Pts',(17.4343438208572,-17.2808977241864,-10.4247632935517));
#83967=CARTESIAN_POINT('Ctrl Pts',(17.4343671095064,-17.2808796123054,-10.4247650761604));
#83968=CARTESIAN_POINT('Ctrl Pts',(17.4343788573469,-17.280870476058,-10.4247659753897));
#83969=CARTESIAN_POINT('Ctrl Pts',(17.434402564613,-17.2808520394157,-10.4247677900471));
#83970=CARTESIAN_POINT('Ctrl Pts',(17.4344145237941,-17.2808427392181,-10.4247687054565));
#83971=CARTESIAN_POINT('Ctrl Pts',(17.4344386581191,-17.2808239712925,-10.4247705528093));
#83972=CARTESIAN_POINT('Ctrl Pts',(17.4344508336627,-17.2808145032613,-10.4247714847833));
#83973=CARTESIAN_POINT('Ctrl Pts',(17.4344754055093,-17.2807953959613,-10.4247733656326));
#83974=CARTESIAN_POINT('Ctrl Pts',(17.4344878019324,-17.2807857566069,-10.4247743145172));
#83975=CARTESIAN_POINT('Ctrl Pts',(17.4345128210006,-17.2807663024365,-10.4247762296059));
#83976=CARTESIAN_POINT('Ctrl Pts',(17.4345254431522,-17.2807564880123,-10.4247771957724));
#83977=CARTESIAN_POINT('Ctrl Pts',(17.4372271946654,-17.2786557752162,-10.4249840025462));
#83978=CARTESIAN_POINT('Ctrl Pts',(17.4399213086497,-17.2765714150477,-10.4251903083905));
#83979=CARTESIAN_POINT('Ctrl Pts',(17.4462368379433,-17.2717095883662,-10.4256741155736));
#83980=CARTESIAN_POINT('Ctrl Pts',(17.4498621993395,-17.2689373342052,-10.425951979191));
#83981=CARTESIAN_POINT('Ctrl Pts',(17.4609904117718,-17.2604846590334,-10.4268052458496));
#83982=CARTESIAN_POINT('Ctrl Pts',(17.4685220801027,-17.2548426156722,-10.4273832307782));
#83983=CARTESIAN_POINT('Ctrl Pts',(17.5765591998817,-17.1750299844123,-10.4356779870282));
#83984=CARTESIAN_POINT('Ctrl Pts',(17.6833880856362,-17.1098547430657,-10.4439142034803));
#83985=CARTESIAN_POINT('Ctrl Pts',(17.8826759478233,-17.0112696685007,-10.4586062915951));
#83986=CARTESIAN_POINT('Ctrl Pts',(17.9729143846822,-16.9741380379784,-10.4650412392758));
#83987=CARTESIAN_POINT('Ctrl Pts',(18.1416604209499,-16.9179686062853,-10.4765055227985));
#83988=CARTESIAN_POINT('Ctrl Pts',(18.2193165345692,-16.8969444210316,-10.4815759029189));
#83989=CARTESIAN_POINT('Ctrl Pts',(18.3170891144227,-16.8763662908325,-10.4877013480118));
#83990=CARTESIAN_POINT('Ctrl Pts',(18.3362445541117,-16.8726105159288,-10.4888895556492));
#83991=CARTESIAN_POINT('Ctrl Pts',(18.3639933366125,-16.8675673497193,-10.4905941701789));
#83992=CARTESIAN_POINT('Ctrl Pts',(18.372546528857,-16.8660671640207,-10.4911173242951));
#83993=CARTESIAN_POINT('Ctrl Pts',(18.3874880658084,-16.8635411573442,-10.4920273312611));
#83994=CARTESIAN_POINT('Ctrl Pts',(18.3938722857777,-16.8624919245277,-10.4924149234685));
#83995=CARTESIAN_POINT('Ctrl Pts',(18.4062270690838,-16.8605195665339,-10.4931626430057));
#83996=CARTESIAN_POINT('Ctrl Pts',(18.4121969636911,-16.859592701026,-10.4935228855141));
#83997=CARTESIAN_POINT('Ctrl Pts',(18.4263967206974,-16.8574503040577,-10.4943772674956));
#83998=CARTESIAN_POINT('Ctrl Pts',(18.4346299808463,-16.8562576969376,-10.4948706781073));
#83999=CARTESIAN_POINT('Ctrl Pts',(18.4639119574695,-16.8521922131341,-10.4966186771941));
#84000=CARTESIAN_POINT('Ctrl Pts',(18.4849970837712,-16.8495876026577,-10.4978648075283));
#84001=CARTESIAN_POINT('Ctrl Pts',(18.6982442863204,-16.8264987417738,-10.5103509151992));
#84002=CARTESIAN_POINT('Ctrl Pts',(18.8923053065221,-16.8320993687426,-10.5206475254935));
#84003=CARTESIAN_POINT('Ctrl Pts',(19.1571395370831,-16.8763546464686,-10.535311059684));
#84004=CARTESIAN_POINT('Ctrl Pts',(19.2306353052451,-16.8927034381921,-10.5394629962477));
#84005=CARTESIAN_POINT('Ctrl Pts',(19.3365015837663,-16.9222503823116,-10.5457590964919));
#84006=CARTESIAN_POINT('Ctrl Pts',(19.3696682606981,-16.9323918157137,-10.5477783634753));
#84007=CARTESIAN_POINT('Ctrl Pts',(19.4095734103534,-16.9456739873161,-10.5502817122309));
#84008=CARTESIAN_POINT('Ctrl Pts',(19.4165657738856,-16.9480420506849,-10.5507231426473));
#84009=CARTESIAN_POINT('Ctrl Pts',(19.427460711142,-16.9517954128764,-10.5514155028952));
#84010=CARTESIAN_POINT('Ctrl Pts',(19.4313719268296,-16.9531556980988,-10.5516649766447));
#84011=CARTESIAN_POINT('Ctrl Pts',(19.4386455321873,-16.9557093388463,-10.5521306772596));
#84012=CARTESIAN_POINT('Ctrl Pts',(19.4420089049835,-16.9568997218985,-10.5523467272029));
#84013=CARTESIAN_POINT('Ctrl Pts',(19.4496413340499,-16.9596227629318,-10.5528386034226));
#84014=CARTESIAN_POINT('Ctrl Pts',(19.4539084644299,-16.9611606353738,-10.5531147359161));
#84015=CARTESIAN_POINT('Ctrl Pts',(19.4668804961102,-16.9658829101426,-10.5539575614396));
#84016=CARTESIAN_POINT('Ctrl Pts',(19.4755693197067,-16.9691107310093,-10.5545267469936));
#84017=CARTESIAN_POINT('Ctrl Pts',(19.5466869728538,-16.9960631127908,-10.5592221120239));
#84018=CARTESIAN_POINT('Ctrl Pts',(19.6079763409848,-17.0226703956028,-10.563499844617));
#84019=CARTESIAN_POINT('Ctrl Pts',(19.7958056823339,-17.1149994914483,-10.5771311150576));
#84020=CARTESIAN_POINT('Ctrl Pts',(19.9170382670057,-17.190629420154,-10.5866767413016));
#84021=CARTESIAN_POINT('Ctrl Pts',(20.1022093346365,-17.3339498669711,-10.6018648834506));
#84022=CARTESIAN_POINT('Ctrl Pts',(20.1709520703969,-17.3946767971232,-10.6076755134377));
#84023=CARTESIAN_POINT('Ctrl Pts',(20.2503104294872,-17.4745257827171,-10.6145874309149));
#84024=CARTESIAN_POINT('Ctrl Pts',(20.2648490943437,-17.4895949668145,-10.6158632641936));
#84025=CARTESIAN_POINT('Ctrl Pts',(20.2852682725264,-17.5113975090061,-10.617669540498));
#84026=CARTESIAN_POINT('Ctrl Pts',(20.2913330592761,-17.5179558804858,-10.6182078991199));
#84027=CARTESIAN_POINT('Ctrl Pts',(20.3017474166265,-17.5293617995574,-10.6191356876734));
#84028=CARTESIAN_POINT('Ctrl Pts',(20.3061164277123,-17.5341913560407,-10.6195259418367));
#84029=CARTESIAN_POINT('Ctrl Pts',(20.3144551459166,-17.5434950103503,-10.6202728057281));
#84030=CARTESIAN_POINT('Ctrl Pts',(20.3184283077977,-17.5479659146936,-10.6206295590185));
#84031=CARTESIAN_POINT('Ctrl Pts',(20.3287454958181,-17.5596751665547,-10.6215583331246));
#84032=CARTESIAN_POINT('Ctrl Pts',(20.3350592468498,-17.5669400984122,-10.6221290883625));
#84033=CARTESIAN_POINT('Ctrl Pts',(20.3565958212548,-17.5920652561579,-10.6240844688312));
#84034=CARTESIAN_POINT('Ctrl Pts',(20.3715714382808,-17.6101357908146,-10.625458948499));
#84035=CARTESIAN_POINT('Ctrl Pts',(20.4912072645767,-17.7594825403026,-10.6365730948589));
#84036=CARTESIAN_POINT('Ctrl Pts',(20.5802124526461,-17.9025326194117,-10.6456351875857));
#84037=CARTESIAN_POINT('Ctrl Pts',(20.7043933598906,-18.1678606626902,-10.6615584261013));
#84038=CARTESIAN_POINT('Ctrl Pts',(20.7472529126862,-18.2855704868649,-10.6683819374743));
#84039=CARTESIAN_POINT('Ctrl Pts',(20.7825424261936,-18.4178607171359,-10.6764615540531));
#84040=CARTESIAN_POINT('Ctrl Pts',(20.7855149006615,-18.4293936059608,-10.6771693176561));
#84041=CARTESIAN_POINT('Ctrl Pts',(20.7896023678436,-18.4458249959643,-10.6781833096697));
#84042=CARTESIAN_POINT('Ctrl Pts',(20.7907975402753,-18.4507035741912,-10.6784850706102));
#84043=CARTESIAN_POINT('Ctrl Pts',(20.7928273553902,-18.4591185503303,-10.6790068518931));
#84044=CARTESIAN_POINT('Ctrl Pts',(20.7936702849524,-18.4626529658149,-10.6792263965169));
#84045=CARTESIAN_POINT('Ctrl Pts',(20.7952870548881,-18.4695102925572,-10.6796531279984));
#84046=CARTESIAN_POINT('Ctrl Pts',(20.7960619635383,-18.472832911623,-10.6798602462165));
#84047=CARTESIAN_POINT('Ctrl Pts',(20.7981311318241,-18.4818029778892,-10.6804203235951));
#84048=CARTESIAN_POINT('Ctrl Pts',(20.7994102334984,-18.4874538402772,-10.6807741385661));
#84049=CARTESIAN_POINT('Ctrl Pts',(20.8040723066368,-18.5084500364147,-10.6820922292244));
#84050=CARTESIAN_POINT('Ctrl Pts',(20.8073074901412,-18.5238272044843,-10.6830644290956));
#84051=CARTESIAN_POINT('Ctrl Pts',(20.8364705749624,-18.6705302663026,-10.6923954376812));
#84052=CARTESIAN_POINT('Ctrl Pts',(20.8500563621851,-18.8039898226102,-10.7012896479728));
#84053=CARTESIAN_POINT('Ctrl Pts',(20.85200493925,-19.0949893046459,-10.7205093060345));
#84054=CARTESIAN_POINT('Ctrl Pts',(20.8355523653503,-19.2518099903764,-10.7307324171897));
#84055=CARTESIAN_POINT('Ctrl Pts',(20.7973240968224,-19.4261680364127,-10.7416955699171));
#84056=CARTESIAN_POINT('Ctrl Pts',(20.7924544485282,-19.4468807841091,-10.7429923041802));
#84057=CARTESIAN_POINT('Ctrl Pts',(20.7850840122204,-19.4762367769593,-10.7448227101385));
#84058=CARTESIAN_POINT('Ctrl Pts',(20.7828392362414,-19.4849424091192,-10.7453645891602));
#84059=CARTESIAN_POINT('Ctrl Pts',(20.778870192563,-19.4999392688035,-10.7462965226963));
#84060=CARTESIAN_POINT('Ctrl Pts',(20.7771721921213,-19.5062372610626,-10.7466874213306));
#84061=CARTESIAN_POINT('Ctrl Pts',(20.7738647143941,-19.5182831212043,-10.7474342079286));
#84062=CARTESIAN_POINT('Ctrl Pts',(20.7722599857531,-19.5240322176176,-10.7477902457368));
#84063=CARTESIAN_POINT('Ctrl Pts',(20.768022622609,-19.5389687456063,-10.7487143097512));
#84064=CARTESIAN_POINT('Ctrl Pts',(20.765352031739,-19.5481453390798,-10.7492810959347));
#84065=CARTESIAN_POINT('Ctrl Pts',(20.7560266021084,-19.5793986564589,-10.7512084953934));
#84066=CARTESIAN_POINT('Ctrl Pts',(20.7490731321349,-19.6013850840226,-10.7525593561758));
#84067=CARTESIAN_POINT('Ctrl Pts',(20.6864103406826,-19.7888132639802,-10.7640423281161));
#84068=CARTESIAN_POINT('Ctrl Pts',(20.6107963541032,-19.94688932184,-10.7734326648572));
#84069=CARTESIAN_POINT('Ctrl Pts',(20.4693507240146,-20.1677007465341,-10.7876988016149));
#84070=CARTESIAN_POINT('Ctrl Pts',(20.4175422226478,-20.238488862108,-10.7924949457549));
#84071=CARTESIAN_POINT('Ctrl Pts',(20.3372095521348,-20.3350585564626,-10.799665664081));
#84072=CARTESIAN_POINT('Ctrl Pts',(20.3121378317858,-20.3635992414914,-10.8018718214812));
#84073=CARTESIAN_POINT('Ctrl Pts',(20.2811592323296,-20.3970068442711,-10.8045824834124));
#84074=CARTESIAN_POINT('Ctrl Pts',(20.275974882188,-20.4025378067928,-10.8050356285985));
#84075=CARTESIAN_POINT('Ctrl Pts',(20.2678831509599,-20.4110781292601,-10.805742364404));
#84076=CARTESIAN_POINT('Ctrl Pts',(20.2649963053727,-20.4141069797807,-10.8059943988872));
#84077=CARTESIAN_POINT('Ctrl Pts',(20.2596342273632,-20.4196995277286,-10.8064623852762));
#84078=CARTESIAN_POINT('Ctrl Pts',(20.257161494037,-20.4222655412884,-10.8066781445864));
#84079=CARTESIAN_POINT('Ctrl Pts',(20.2515672091084,-20.4280416031312,-10.8071661514529));
#84080=CARTESIAN_POINT('Ctrl Pts',(20.248441963686,-20.4312479799241,-10.8074386851726));
#84081=CARTESIAN_POINT('Ctrl Pts',(20.2392187044678,-20.4406508099476,-10.808242655362));
#84082=CARTESIAN_POINT('Ctrl Pts',(20.2330927510674,-20.4468195543203,-10.8087762132711));
#84083=CARTESIAN_POINT('Ctrl Pts',(20.1894856228256,-20.4901936433746,-10.8125701295656));
#84084=CARTESIAN_POINT('Ctrl Pts',(20.1506648572465,-20.5260196174447,-10.8159256372911));
#84085=CARTESIAN_POINT('Ctrl Pts',(20.0984360446275,-20.5707209440942,-10.8203670826831));
#84086=CARTESIAN_POINT('Ctrl Pts',(20.0862062638983,-20.5809510171277,-10.821402165138));
#84087=CARTESIAN_POINT('Ctrl Pts',(19.9575080993183,-20.6861575006348,-10.8322348412543));
#84088=CARTESIAN_POINT('Ctrl Pts',(19.831354046004,-20.7686160568631,-10.8423075176814));
#84089=CARTESIAN_POINT('Ctrl Pts',(19.6427152026762,-20.8650379480273,-10.8559924833463));
#84090=CARTESIAN_POINT('Ctrl Pts',(19.5867096702835,-20.8906502639685,-10.8599069390703));
#84091=CARTESIAN_POINT('Ctrl Pts',(19.4952389926382,-20.9277490093902,-10.8660569255437));
#84092=CARTESIAN_POINT('Ctrl Pts',(19.4604517634608,-20.9408029217722,-10.8683418998437));
#84093=CARTESIAN_POINT('Ctrl Pts',(19.4148238994026,-20.9565676695649,-10.8712714745627));
#84094=CARTESIAN_POINT('Ctrl Pts',(19.4042819849423,-20.9601172256424,-10.8719437311783));
#84095=CARTESIAN_POINT('Ctrl Pts',(19.3870920281101,-20.9657547880979,-10.8730326028818));
#84096=CARTESIAN_POINT('Ctrl Pts',(19.3804608932809,-20.9678933153896,-10.8734508788304));
#84097=CARTESIAN_POINT('Ctrl Pts',(19.367688445844,-20.9719428999078,-10.8742531913098));
#84098=CARTESIAN_POINT('Ctrl Pts',(19.3615487544839,-20.9738587802908,-10.874637382709));
#84099=CARTESIAN_POINT('Ctrl Pts',(19.347471098241,-20.9781813869704,-10.8755149562976));
#84100=CARTESIAN_POINT('Ctrl Pts',(19.3395274966263,-20.9805695095562,-10.8760077247103));
#84101=CARTESIAN_POINT('Ctrl Pts',(19.3183871484546,-20.9867897909643,-10.87731283719));
#84102=CARTESIAN_POINT('Ctrl Pts',(19.3051666407347,-20.9905402901307,-10.8781225199301));
#84103=CARTESIAN_POINT('Ctrl Pts',(19.2041077209126,-21.0181491759718,-10.8842643076848));
#84104=CARTESIAN_POINT('Ctrl Pts',(19.1148437982584,-21.0364506741887,-10.8894106888243));
#84105=CARTESIAN_POINT('Ctrl Pts',(18.8852420271653,-21.0682770240549,-10.9022378076773));
#84106=CARTESIAN_POINT('Ctrl Pts',(18.7442412702683,-21.0736492610361,-10.9097208562789));
#84107=CARTESIAN_POINT('Ctrl Pts',(18.5500364719464,-21.0616784187743,-10.9204806198787));
#84108=CARTESIAN_POINT('Ctrl Pts',(18.4964676334484,-21.0563201251308,-10.9235000316635));
#84109=CARTESIAN_POINT('Ctrl Pts',(18.4154529922025,-21.0450837387864,-10.9282206389264));
#84110=CARTESIAN_POINT('Ctrl Pts',(18.3878213029995,-21.0406914258585,-10.9298583197723));
#84111=CARTESIAN_POINT('Ctrl Pts',(18.3534916153607,-21.0345345188211,-10.931936547882));
#84112=CARTESIAN_POINT('Ctrl Pts',(18.3467030292591,-21.0332827069673,-10.9323496466053));
#84113=CARTESIAN_POINT('Ctrl Pts',(18.3359559927064,-21.0312465587741,-10.933007185181));
#84114=CARTESIAN_POINT('Ctrl Pts',(18.3319933853742,-21.0304840545665,-10.9332503989365));
#84115=CARTESIAN_POINT('Ctrl Pts',(18.3245141947058,-21.0290226840651,-10.9337109442059));
#84116=CARTESIAN_POINT('Ctrl Pts',(18.3209971978838,-21.0283262122265,-10.9339281385505));
#84117=CARTESIAN_POINT('Ctrl Pts',(18.3129476165207,-21.0267108904733,-10.9344266719472));
#84118=CARTESIAN_POINT('Ctrl Pts',(18.3084162667374,-21.0257861205361,-10.9347083455272));
#84119=CARTESIAN_POINT('Ctrl Pts',(18.2963676932262,-21.0232860629597,-10.9354599845175));
#84120=CARTESIAN_POINT('Ctrl Pts',(18.2888560309,-21.0216847183123,-10.9359313794122));
#84121=CARTESIAN_POINT('Ctrl Pts',(18.2355596493348,-21.0100193747706,-10.9392950048503));
#84122=CARTESIAN_POINT('Ctrl Pts',(18.190115148787,-20.998478699073,-10.942262682062));
#84123=CARTESIAN_POINT('Ctrl Pts',(18.1409667008456,-20.9842448129227,-10.9455548968351));
#84124=CARTESIAN_POINT('Ctrl Pts',(18.1368419365551,-20.9830366122723,-10.9458318392832));
#84125=CARTESIAN_POINT('Ctrl Pts',(18.1279297894155,-20.9803966251375,-10.9464315701298));
#84126=CARTESIAN_POINT('Ctrl Pts',(18.1231437445308,-20.978960434628,-10.9467544893002));
#84127=CARTESIAN_POINT('Ctrl Pts',(18.094639858601,-20.9702969009925,-10.9486825761938));
#84128=CARTESIAN_POINT('Ctrl Pts',(18.0710459346062,-20.9626704396908,-10.9502987800727));
#84129=CARTESIAN_POINT('Ctrl Pts',(18.0104709079159,-20.9419081673084,-10.9544925318567));
#84130=CARTESIAN_POINT('Ctrl Pts',(17.9737113750762,-20.9281553479168,-10.9570806034525));
#84131=CARTESIAN_POINT('Ctrl Pts',(17.836096163845,-20.8722611214751,-10.9668924806917));
#84132=CARTESIAN_POINT('Ctrl Pts',(17.7381654037347,-20.8233500470731,-10.9741188246851));
#84133=CARTESIAN_POINT('Ctrl Pts',(17.5972934615871,-20.7387880667882,-10.9846789172014));
#84134=CARTESIAN_POINT('Ctrl Pts',(17.551260073831,-20.708656037397,-10.9881610876758));
#84135=CARTESIAN_POINT('Ctrl Pts',(17.4785408295698,-20.6569001987935,-10.9937088594141));
#84136=CARTESIAN_POINT('Ctrl Pts',(17.4511174735847,-20.6363619133967,-10.9958127306643));
#84137=CARTESIAN_POINT('Ctrl Pts',(17.4157162859835,-20.6084823429287,-10.998545997722));
#84138=CARTESIAN_POINT('Ctrl Pts',(17.4072804169872,-20.6017335717931,-10.9991986653204));
#84139=CARTESIAN_POINT('Ctrl Pts',(17.3935441170201,-20.5905708991804,-11.000263756248));
#84140=CARTESIAN_POINT('Ctrl Pts',(17.3882130199049,-20.5861952061532,-11.000677706756));
#84141=CARTESIAN_POINT('Ctrl Pts',(17.3779321910357,-20.5776724126579,-11.0014771761271));
#84142=CARTESIAN_POINT('Ctrl Pts',(17.3729798695196,-20.5735285694797,-11.0018628208234));
#84143=CARTESIAN_POINT('Ctrl Pts',(17.3615850294236,-20.563904984718,-11.0027514443956));
#84144=CARTESIAN_POINT('Ctrl Pts',(17.3551562068402,-20.558409141051,-11.0032537562283));
#84145=CARTESIAN_POINT('Ctrl Pts',(17.3379467274318,-20.5435177509331,-11.0046011425119));
#84146=CARTESIAN_POINT('Ctrl Pts',(17.3272279300886,-20.5340511526633,-11.0054432701842));
#84147=CARTESIAN_POINT('Ctrl Pts',(17.2292160839547,-20.4457055177877,-11.0131733402474));
#84148=CARTESIAN_POINT('Ctrl Pts',(17.1485394364045,-20.3597822811603,-11.0197398132545));
#84149=CARTESIAN_POINT('Ctrl Pts',(16.9737390657472,-20.1394082055912,-11.0351343331842));
#84150=CARTESIAN_POINT('Ctrl Pts',(16.887280690716,-19.9998894240454,-11.0437794300367));
#84151=CARTESIAN_POINT('Ctrl Pts',(16.8045807977523,-19.8237747371058,-11.0549699554387));
#84152=CARTESIAN_POINT('Ctrl Pts',(16.7920251456033,-19.7954352889854,-11.0567798462889));
#84153=CARTESIAN_POINT('Ctrl Pts',(16.7773512483217,-19.7602484435683,-11.0590503268335));
#84154=CARTESIAN_POINT('Ctrl Pts',(16.7746389829561,-19.7536509749048,-11.0594770317163));
#84155=CARTESIAN_POINT('Ctrl Pts',(16.7704255513855,-19.7432528562106,-11.0601513013589));
#84156=CARTESIAN_POINT('Ctrl Pts',(16.7689019295681,-19.7394612819996,-11.0603975316799));
#84157=CARTESIAN_POINT('Ctrl Pts',(16.7660657190618,-19.7323438027719,-11.0608604760077));
#84158=CARTESIAN_POINT('Ctrl Pts',(16.7647505755928,-19.7290189755786,-11.0610770333961));
#84159=CARTESIAN_POINT('Ctrl Pts',(16.7617562471679,-19.7213925544098,-11.0615744439044));
#84160=CARTESIAN_POINT('Ctrl Pts',(16.7600827142915,-19.7170887998233,-11.061855631285));
#84161=CARTESIAN_POINT('Ctrl Pts',(16.7549425676338,-19.7037409743647,-11.0627291480247));
#84162=CARTESIAN_POINT('Ctrl Pts',(16.7515239884571,-19.6946787115692,-11.0633242370727));
#84163=CARTESIAN_POINT('Ctrl Pts',(16.7472469472791,-19.6831007927047,-11.0640868106714));
#84164=CARTESIAN_POINT('Ctrl Pts',(16.7463308324829,-19.6806064376839,-11.0642512349997));
#84165=CARTESIAN_POINT('Ctrl Pts',(16.745419450227,-19.678110457895,-11.0644158965713));
#84166=CARTESIAN_POINT('',(16.617000600774,-18.9535948907958,-10.0879364327122));
#84167=CARTESIAN_POINT('Ctrl Pts',(16.7454194496957,-19.67811045644,-10.8441190240937));
#84168=CARTESIAN_POINT('Ctrl Pts',(16.7463456800211,-19.6806471002713,-10.843971851373));
#84169=CARTESIAN_POINT('Ctrl Pts',(16.7472767931095,-19.6831820516202,-10.8438247185697));
#84170=CARTESIAN_POINT('Ctrl Pts',(16.8056499896822,-19.8411680552622,-10.8346510169722));
#84171=CARTESIAN_POINT('Ctrl Pts',(16.8811330167863,-19.9893140728775,-10.8258505642691));
#84172=CARTESIAN_POINT('Ctrl Pts',(16.9808578145588,-20.1387506075834,-10.8152891817525));
#84173=CARTESIAN_POINT('Ctrl Pts',(16.9887344675016,-20.1503041036104,-10.81446052175));
#84174=CARTESIAN_POINT('Ctrl Pts',(16.9998805544108,-20.1663101930112,-10.8132942201619));
#84175=CARTESIAN_POINT('Ctrl Pts',(17.0030540337989,-20.1708295848692,-10.8129628507967));
#84176=CARTESIAN_POINT('Ctrl Pts',(17.0081863136465,-20.1780780581372,-10.8124279704154));
#84177=CARTESIAN_POINT('Ctrl Pts',(17.0101340155851,-20.1808150194652,-10.8122252173516));
#84178=CARTESIAN_POINT('Ctrl Pts',(17.0142251835164,-20.1865351653663,-10.8117997947541));
#84179=CARTESIAN_POINT('Ctrl Pts',(17.0163699018095,-20.1895174095777,-10.8115770358813));
#84180=CARTESIAN_POINT('Ctrl Pts',(17.0215923838734,-20.1967395736061,-10.8110352681897));
#84181=CARTESIAN_POINT('Ctrl Pts',(17.0246781358097,-20.2009736639017,-10.8107157114476));
#84182=CARTESIAN_POINT('Ctrl Pts',(17.0356087281591,-20.215855611602,-10.8095858154991));
#84183=CARTESIAN_POINT('Ctrl Pts',(17.0435374145915,-20.2264411113385,-10.8087699389654));
#84184=CARTESIAN_POINT('Ctrl Pts',(17.0915651139364,-20.2893255989126,-10.8038531908166));
#84185=CARTESIAN_POINT('Ctrl Pts',(17.1339858546124,-20.3397986782992,-10.7996154560109));
#84186=CARTESIAN_POINT('Ctrl Pts',(17.2439182575073,-20.4588479826325,-10.7890378176297));
#84187=CARTESIAN_POINT('Ctrl Pts',(17.3138862660322,-20.5249625715988,-10.782642147312));
#84188=CARTESIAN_POINT('Ctrl Pts',(17.4967378907325,-20.6755654973935,-10.7670586086159));
#84189=CARTESIAN_POINT('Ctrl Pts',(17.6140381141675,-20.7539972808021,-10.75801007058));
#84190=CARTESIAN_POINT('Ctrl Pts',(17.7508859013276,-20.826934621051,-10.7485414219303));
#84191=CARTESIAN_POINT('Ctrl Pts',(17.7635632873743,-20.8335275088946,-10.7476734914909));
#84192=CARTESIAN_POINT('Ctrl Pts',(17.7838464468635,-20.8438162438814,-10.7462992412623));
#84193=CARTESIAN_POINT('Ctrl Pts',(17.7914091200073,-20.8475956613542,-10.7457899937914));
#84194=CARTESIAN_POINT('Ctrl Pts',(17.8047871228581,-20.8541814103034,-10.7448946309647));
#84195=CARTESIAN_POINT('Ctrl Pts',(17.8105929931825,-20.8570066115222,-10.744507859552));
#84196=CARTESIAN_POINT('Ctrl Pts',(17.8226282410899,-20.8627951490027,-10.7437097879834));
#84197=CARTESIAN_POINT('Ctrl Pts',(17.8288593661852,-20.8657546914745,-10.7432986232449));
#84198=CARTESIAN_POINT('Ctrl Pts',(17.8448911678738,-20.8732733590284,-10.7422458852346));
#84199=CARTESIAN_POINT('Ctrl Pts',(17.8547125738495,-20.8777880112437,-10.7416058534271));
#84200=CARTESIAN_POINT('Ctrl Pts',(17.8958499548665,-20.8963175099897,-10.738944964163));
#84201=CARTESIAN_POINT('Ctrl Pts',(17.9274707408071,-20.9096457362182,-10.7369476405012));
#84202=CARTESIAN_POINT('Ctrl Pts',(18.0106938037344,-20.9423654298589,-10.731802945253));
#84203=CARTESIAN_POINT('Ctrl Pts',(18.0627549184162,-20.9605211186356,-10.7286949750687));
#84204=CARTESIAN_POINT('Ctrl Pts',(18.2200494114054,-21.008575261138,-10.7195498472431));
#84205=CARTESIAN_POINT('Ctrl Pts',(18.3269517750913,-21.0323748791323,-10.7136614166043));
#84206=CARTESIAN_POINT('Ctrl Pts',(18.4810888454796,-21.0543492181285,-10.7051846664263));
#84207=CARTESIAN_POINT('Ctrl Pts',(18.5271649116022,-21.0593811436068,-10.7026508060785));
#84208=CARTESIAN_POINT('Ctrl Pts',(18.5947027529102,-21.064520557752,-10.6988935424562));
#84209=CARTESIAN_POINT('Ctrl Pts',(18.6160609289931,-21.0658205133526,-10.69769902599));
#84210=CARTESIAN_POINT('Ctrl Pts',(18.6892331614252,-21.0691616880528,-10.693574458071));
#84211=CARTESIAN_POINT('Ctrl Pts',(18.7410966719304,-21.069622812678,-10.6905959184217));
#84212=CARTESIAN_POINT('Ctrl Pts',(18.8015718440414,-21.0679390251815,-10.6870052830929));
#84213=CARTESIAN_POINT('Ctrl Pts',(18.8102219599894,-21.067645083519,-10.6864888811617));
#84214=CARTESIAN_POINT('Ctrl Pts',(18.8233354723751,-21.0671189439723,-10.6857014274819));
#84215=CARTESIAN_POINT('Ctrl Pts',(18.8278004568098,-21.0669256363369,-10.6854325017877));
#84216=CARTESIAN_POINT('Ctrl Pts',(18.8358239962299,-21.0665528060063,-10.6849477394157));
#84217=CARTESIAN_POINT('Ctrl Pts',(18.8393827362904,-21.066378436842,-10.6847321940829));
#84218=CARTESIAN_POINT('Ctrl Pts',(18.8471262713922,-21.0659794249753,-10.6842620089058));
#84219=CARTESIAN_POINT('Ctrl Pts',(18.8513107909387,-21.0657513430214,-10.6840071838548));
#84220=CARTESIAN_POINT('Ctrl Pts',(18.8630928885763,-21.0650740525226,-10.6832876506464));
#84221=CARTESIAN_POINT('Ctrl Pts',(18.8706886711193,-21.0645963004026,-10.6828213887988));
#84222=CARTESIAN_POINT('Ctrl Pts',(18.9167087806202,-21.0614525456349,-10.6799826793448));
#84223=CARTESIAN_POINT('Ctrl Pts',(18.9550544817785,-21.0577794342677,-10.6775591194044));
#84224=CARTESIAN_POINT('Ctrl Pts',(19.0823758889858,-21.0420676956464,-10.6693637562636));
#84225=CARTESIAN_POINT('Ctrl Pts',(19.1706810236437,-21.0254166085174,-10.6634408191298));
#84226=CARTESIAN_POINT('Ctrl Pts',(19.4238618436034,-20.9607817782371,-10.6461738940246));
#84227=CARTESIAN_POINT('Ctrl Pts',(19.5843274020447,-20.8982987635037,-10.6349279584136));
#84228=CARTESIAN_POINT('Ctrl Pts',(19.7560011913052,-20.806115288656,-10.6229309460918));
#84229=CARTESIAN_POINT('Ctrl Pts',(19.7763099133725,-20.7947750950297,-10.6215108768762));
#84230=CARTESIAN_POINT('Ctrl Pts',(19.8047233092177,-20.7782892887542,-10.6195221811033));
#84231=CARTESIAN_POINT('Ctrl Pts',(19.8129856342374,-20.7734200440766,-10.6189436521902));
#84232=CARTESIAN_POINT('Ctrl Pts',(19.8263413820472,-20.7654263159396,-10.6180080118978));
#84233=CARTESIAN_POINT('Ctrl Pts',(19.8314550974713,-20.7623361589624,-10.6176496563862));
#84234=CARTESIAN_POINT('Ctrl Pts',(19.8421196515338,-20.7558299026823,-10.6169020462657));
#84235=CARTESIAN_POINT('Ctrl Pts',(19.8476679415611,-20.7524097304032,-10.6165129460599));
#84236=CARTESIAN_POINT('Ctrl Pts',(19.8608074056511,-20.744226097483,-10.6155910674706));
#84237=CARTESIAN_POINT('Ctrl Pts',(19.8683843405866,-20.7394399250109,-10.6150591337573));
#84238=CARTESIAN_POINT('Ctrl Pts',(19.8937052192919,-20.7232194622086,-10.6132801928249));
#84239=CARTESIAN_POINT('Ctrl Pts',(19.9113088502268,-20.7115677019112,-10.6120412819522));
#84240=CARTESIAN_POINT('Ctrl Pts',(20.0055364049833,-20.6471516274508,-10.6053929064818));
#84241=CARTESIAN_POINT('Ctrl Pts',(20.0787974964785,-20.5896405171448,-10.600169027024));
#84242=CARTESIAN_POINT('Ctrl Pts',(20.2631896580524,-20.4241436645837,-10.5865244081878));
#84243=CARTESIAN_POINT('Ctrl Pts',(20.3666490248463,-20.3084950083429,-10.5783424624455));
#84244=CARTESIAN_POINT('Ctrl Pts',(20.4877603804611,-20.1389672088419,-10.5666285142275));
#84245=CARTESIAN_POINT('Ctrl Pts',(20.5172703927468,-20.0941524849342,-10.5635510937905));
#84246=CARTESIAN_POINT('Ctrl Pts',(20.5495710881144,-20.0407915516664,-10.5598496972577));
#84247=CARTESIAN_POINT('Ctrl Pts',(20.5540514973316,-20.0332853277824,-10.5593281942504));
#84248=CARTESIAN_POINT('Ctrl Pts',(20.5607614694286,-20.0218839538951,-10.5585344814504));
#84249=CARTESIAN_POINT('Ctrl Pts',(20.5630254087612,-20.018009002891,-10.5582644487195));
#84250=CARTESIAN_POINT('Ctrl Pts',(20.5670652343483,-20.011043696335,-10.557778511095));
#84251=CARTESIAN_POINT('Ctrl Pts',(20.5688456514959,-20.0079560308161,-10.5575629038588));
#84252=CARTESIAN_POINT('Ctrl Pts',(20.5726953256614,-20.0012406497307,-10.5570935438061));
#84253=CARTESIAN_POINT('Ctrl Pts',(20.5747616206543,-19.9976113507834,-10.5568396110304));
#84254=CARTESIAN_POINT('Ctrl Pts',(20.5805304195922,-19.9874087726088,-10.5561250606686));
#84255=CARTESIAN_POINT('Ctrl Pts',(20.5842085011695,-19.9808218578252,-10.555662922932));
#84256=CARTESIAN_POINT('Ctrl Pts',(20.6058848281407,-19.941510495461,-10.5529006498017));
#84257=CARTESIAN_POINT('Ctrl Pts',(20.62304856624,-19.9083362113267,-10.5505524815628));
#84258=CARTESIAN_POINT('Ctrl Pts',(20.6764341811795,-19.798101182503,-10.5427357876341));
#84259=CARTESIAN_POINT('Ctrl Pts',(20.7088849599637,-19.7193104245221,-10.5371299076634));
#84260=CARTESIAN_POINT('Ctrl Pts',(20.7942907005149,-19.4702879052617,-10.5197385422854));
#84261=CARTESIAN_POINT('Ctrl Pts',(20.8305934425447,-19.2951334505474,-10.5080322030861));
#84262=CARTESIAN_POINT('Ctrl Pts',(20.846303571535,-19.094764425315,-10.4956637956596));
#84263=CARTESIAN_POINT('Ctrl Pts',(20.8477177020219,-19.0720233280426,-10.494273165356));
#84264=CARTESIAN_POINT('Ctrl Pts',(20.849201512472,-19.0397612553451,-10.4923182409659));
#84265=CARTESIAN_POINT('Ctrl Pts',(20.8495744870978,-19.0302564403979,-10.4917444932049));
#84266=CARTESIAN_POINT('Ctrl Pts',(20.8500769629108,-19.0147918458448,-10.4908144815772));
#84267=CARTESIAN_POINT('Ctrl Pts',(20.8502453729272,-19.008833542559,-10.4904570029324));
#84268=CARTESIAN_POINT('Ctrl Pts',(20.8505455421904,-18.9963464602995,-10.4897095543487));
#84269=CARTESIAN_POINT('Ctrl Pts',(20.8506722633026,-18.9898176142333,-10.4893197461409));
#84270=CARTESIAN_POINT('Ctrl Pts',(20.8509022301395,-18.9742594753132,-10.4883931576885));
#84271=CARTESIAN_POINT('Ctrl Pts',(20.8509779193418,-18.965229855517,-10.4878572456708));
#84272=CARTESIAN_POINT('Ctrl Pts',(20.8510385074532,-18.934690040024,-10.4860507794607));
#84273=CARTESIAN_POINT('Ctrl Pts',(20.8507533513592,-18.9131802055577,-10.4847886732546));
#84274=CARTESIAN_POINT('Ctrl Pts',(20.8450116479682,-18.7117574967599,-10.4730565259586));
#84275=CARTESIAN_POINT('Ctrl Pts',(20.8169604240109,-18.5332286439743,-10.4633886770937));
#84276=CARTESIAN_POINT('Ctrl Pts',(20.7331466816762,-18.2452622428535,-10.4470646166408));
#84277=CARTESIAN_POINT('Ctrl Pts',(20.6899232829007,-18.1332073185101,-10.4404840010678));
#84278=CARTESIAN_POINT('Ctrl Pts',(20.6332945078128,-18.0168743813086,-10.4328161849434));
#84279=CARTESIAN_POINT('Ctrl Pts',(20.6290720821249,-18.0083468083841,-10.432248994846));
#84280=CARTESIAN_POINT('Ctrl Pts',(20.6227304272447,-17.9957534881795,-10.4314033536339));
#84281=CARTESIAN_POINT('Ctrl Pts',(20.6206551817095,-17.9916655569072,-10.4311275871715));
#84282=CARTESIAN_POINT('Ctrl Pts',(20.6169393466316,-17.9844044348876,-10.4306354555728));
#84283=CARTESIAN_POINT('Ctrl Pts',(20.6153039880556,-17.9812286237139,-10.4304194206636));
#84284=CARTESIAN_POINT('Ctrl Pts',(20.6117708027984,-17.9744097559684,-10.4299538490456));
#84285=CARTESIAN_POINT('Ctrl Pts',(20.6098704367621,-17.9707681329637,-10.4297041576473));
#84286=CARTESIAN_POINT('Ctrl Pts',(20.6045957604759,-17.9607317313824,-10.4290131415603));
#84287=CARTESIAN_POINT('Ctrl Pts',(20.6011993056273,-17.9543487437641,-10.4285704506624));
#84288=CARTESIAN_POINT('Ctrl Pts',(20.5824161322064,-17.9194812725726,-10.426135084562));
#84289=CARTESIAN_POINT('Ctrl Pts',(20.5664111408816,-17.891336874562,-10.4241064343963));
#84290=CARTESIAN_POINT('Ctrl Pts',(20.4660460361725,-17.7239028978663,-10.4117039053007));
#84291=CARTESIAN_POINT('Ctrl Pts',(20.3664914526004,-17.594363255682,-10.4007374961109));
#84292=CARTESIAN_POINT('Ctrl Pts',(20.1716622478777,-17.3936422461894,-10.3824656027845));
#84293=CARTESIAN_POINT('Ctrl Pts',(20.0834341901537,-17.3166447432572,-10.3750198855405));
#84294=CARTESIAN_POINT('Ctrl Pts',(19.9777935127396,-17.2388536621923,-10.3670094790559));
#84295=CARTESIAN_POINT('Ctrl Pts',(19.966216060809,-17.2305075451167,-10.3661425986559));
#84296=CARTESIAN_POINT('Ctrl Pts',(19.9476512198721,-17.2174075095098,-10.3647696915688));
#84297=CARTESIAN_POINT('Ctrl Pts',(19.9407183925265,-17.2125773613254,-10.3642607460972));
#84298=CARTESIAN_POINT('Ctrl Pts',(19.9284377145922,-17.2041300894364,-10.3633657344842));
#84299=CARTESIAN_POINT('Ctrl Pts',(19.9231019223148,-17.2004957042379,-10.362979013906));
#84300=CARTESIAN_POINT('Ctrl Pts',(19.9120289162187,-17.1930274349134,-10.3621808749664));
#84301=CARTESIAN_POINT('Ctrl Pts',(19.9062894096267,-17.1891970745472,-10.3617695928719));
#84302=CARTESIAN_POINT('Ctrl Pts',(19.8915035832794,-17.1794336434102,-10.3607161975162));
#84303=CARTESIAN_POINT('Ctrl Pts',(19.8824302564333,-17.1735416826635,-10.3600756294999));
#84304=CARTESIAN_POINT('Ctrl Pts',(19.8443282302194,-17.1492124946661,-10.3574095230887));
#84305=CARTESIAN_POINT('Ctrl Pts',(19.8148966791519,-17.1314137935271,-10.3554076364386));
#84306=CARTESIAN_POINT('Ctrl Pts',(19.7370493198039,-17.0868892843295,-10.3502485244327));
#84307=CARTESIAN_POINT('Ctrl Pts',(19.6879962624945,-17.0613287695323,-10.3471309907069));
#84308=CARTESIAN_POINT('Ctrl Pts',(19.4673567208315,-16.9571345621667,-10.333565480744));
#84309=CARTESIAN_POINT('Ctrl Pts',(19.2867325213103,-16.8997395542983,-10.323717755979));
#84310=CARTESIAN_POINT('Ctrl Pts',(19.0604234464957,-16.8599132088181,-10.3106505323397));
#84311=CARTESIAN_POINT('Ctrl Pts',(19.0197350572528,-16.8539689264304,-10.308270138831));
#84312=CARTESIAN_POINT('Ctrl Pts',(18.9715618323872,-16.8483583972142,-10.3053884392312));
#84313=CARTESIAN_POINT('Ctrl Pts',(18.9642168017775,-16.8475419135218,-10.3049473304845));
#84314=CARTESIAN_POINT('Ctrl Pts',(18.9523055510701,-16.8462809462173,-10.3042289718892));
#84315=CARTESIAN_POINT('Ctrl Pts',(18.9477418248774,-16.8458128101993,-10.3039530184238));
#84316=CARTESIAN_POINT('Ctrl Pts',(18.939621626224,-16.8450065235706,-10.3034606820463));
#84317=CARTESIAN_POINT('Ctrl Pts',(18.9360657836174,-16.8446625372875,-10.3032446304212));
#84318=CARTESIAN_POINT('Ctrl Pts',(18.9284215214995,-16.8439425700486,-10.3027791697893));
#84319=CARTESIAN_POINT('Ctrl Pts',(18.9243329342682,-16.8435694866877,-10.3025296068684));
#84320=CARTESIAN_POINT('Ctrl Pts',(18.9130503213187,-16.8425730338913,-10.3018393000788));
#84321=CARTESIAN_POINT('Ctrl Pts',(18.9058542301965,-16.8419745823775,-10.3013971945268));
#84322=CARTESIAN_POINT('Ctrl Pts',(18.8665155855769,-16.8389056173192,-10.2989708999703));
#84323=CARTESIAN_POINT('Ctrl Pts',(18.8343247265084,-16.8371328794595,-10.296951044929));
#84324=CARTESIAN_POINT('Ctrl Pts',(18.6392355953626,-16.8308532261554,-10.2845514364748));
#84325=CARTESIAN_POINT('Ctrl Pts',(18.4763071486216,-16.8444331058325,-10.2735769198782));
#84326=CARTESIAN_POINT('Ctrl Pts',(18.201972448026,-16.8996123972514,-10.2552981298976));
#84327=CARTESIAN_POINT('Ctrl Pts',(18.0894856773053,-16.9321095838726,-10.2478531342966));
#84328=CARTESIAN_POINT('Ctrl Pts',(17.9668770166934,-16.9788259451453,-10.239841513944));
#84329=CARTESIAN_POINT('Ctrl Pts',(17.9535647796046,-16.9840532515357,-10.2389728125279));
#84330=CARTESIAN_POINT('Ctrl Pts',(17.93246527165,-16.9925861550501,-10.2375975762118));
#84331=CARTESIAN_POINT('Ctrl Pts',(17.9246432569934,-16.9958041503149,-10.2370881070898));
#84332=CARTESIAN_POINT('Ctrl Pts',(17.910883813538,-17.0015614749432,-10.2361924864194));
#84333=CARTESIAN_POINT('Ctrl Pts',(17.904938363605,-17.0040812386209,-10.2358056776252));
#84334=CARTESIAN_POINT('Ctrl Pts',(17.893529214847,-17.0089782912008,-10.2350637299531));
#84335=CARTESIAN_POINT('Ctrl Pts',(17.8880638490885,-17.0113515178532,-10.2347084573019));
#84336=CARTESIAN_POINT('Ctrl Pts',(17.8736594437266,-17.0176787583741,-10.2337724496465));
#84337=CARTESIAN_POINT('Ctrl Pts',(17.8647375755608,-17.0216716909042,-10.2331930501737));
#84338=CARTESIAN_POINT('Ctrl Pts',(17.8316970723038,-17.0367343119883,-10.2310483576716));
#84339=CARTESIAN_POINT('Ctrl Pts',(17.8077589493055,-17.0481956933715,-10.2294965538034));
#84340=CARTESIAN_POINT('Ctrl Pts',(17.7489355835763,-17.0777320697137,-10.2256835427367));
#84341=CARTESIAN_POINT('Ctrl Pts',(17.7143254322945,-17.0963340230601,-10.2234404015519));
#84342=CARTESIAN_POINT('Ctrl Pts',(17.5863677572753,-17.1697692514696,-10.2151165562411));
#84343=CARTESIAN_POINT('Ctrl Pts',(17.4967503337795,-17.2307732200334,-10.2092331185111));
#84344=CARTESIAN_POINT('Ctrl Pts',(17.305801030502,-17.3834060554229,-10.1959580002686));
#84345=CARTESIAN_POINT('Ctrl Pts',(17.2078821415528,-17.478503047627,-10.1886008824204));
#84346=CARTESIAN_POINT('Ctrl Pts',(17.1096885973165,-17.5942278921786,-10.1797012658975));
#84347=CARTESIAN_POINT('Ctrl Pts',(17.0997222590636,-17.6062404140771,-10.178777868324));
#84348=CARTESIAN_POINT('Ctrl Pts',(17.0862501024277,-17.6228488952362,-10.1774999990982));
#84349=CARTESIAN_POINT('Ctrl Pts',(17.0826286489866,-17.6273509734594,-10.1771534885434));
#84350=CARTESIAN_POINT('Ctrl Pts',(17.076900114816,-17.6345325090898,-10.1766004609545));
#84351=CARTESIAN_POINT('Ctrl Pts',(17.0747809665971,-17.6372023661811,-10.1763948008226));
#84352=CARTESIAN_POINT('Ctrl Pts',(17.0704149452737,-17.642730362687,-10.1759688203684));
#84353=CARTESIAN_POINT('Ctrl Pts',(17.0681689900703,-17.6455891675752,-10.1757484351316));
#84354=CARTESIAN_POINT('Ctrl Pts',(17.0628305414498,-17.65242045828,-10.1752216228868));
#84355=CARTESIAN_POINT('Ctrl Pts',(17.0597448423315,-17.6563982053628,-10.1749147191133));
#84356=CARTESIAN_POINT('Ctrl Pts',(17.0493660199558,-17.669876447815,-10.173874407744));
#84357=CARTESIAN_POINT('Ctrl Pts',(17.0421394977139,-17.6794276148764,-10.1731365460881));
#84358=CARTESIAN_POINT('Ctrl Pts',(16.9597945784962,-17.7902026100249,-10.1645761939436));
#84359=CARTESIAN_POINT('Ctrl Pts',(16.8937878918033,-17.8978696484181,-10.1562461149533));
#84360=CARTESIAN_POINT('Ctrl Pts',(16.8040458319401,-18.0786648961684,-10.1429073852356));
#84361=CARTESIAN_POINT('Ctrl Pts',(16.774007504723,-18.1483410710766,-10.1379034961777));
#84362=CARTESIAN_POINT('Ctrl Pts',(16.7335752732272,-18.2579732852734,-10.1303131054882));
#84363=CARTESIAN_POINT('Ctrl Pts',(16.7205007736768,-18.2968715188803,-10.127672050771));
#84364=CARTESIAN_POINT('Ctrl Pts',(16.7056936910043,-18.3455679011222,-10.1244341607967));
#84365=CARTESIAN_POINT('Ctrl Pts',(16.7028889806927,-18.3550289742907,-10.1238082280434));
#84366=CARTESIAN_POINT('Ctrl Pts',(16.6846210484773,-18.4182712229377,-10.119645304547));
#84367=CARTESIAN_POINT('Ctrl Pts',(16.6712283446651,-18.472631128594,-10.116169486635));
#84368=CARTESIAN_POINT('Ctrl Pts',(16.6575926819898,-18.5392454571761,-10.1120304203273));
#84369=CARTESIAN_POINT('Ctrl Pts',(16.6552811241882,-18.5510492453933,-10.1113014880045));
#84370=CARTESIAN_POINT('Ctrl Pts',(16.6516247783754,-18.570602205829,-10.1101012830394));
#84371=CARTESIAN_POINT('Ctrl Pts',(16.650222373548,-18.5783401986623,-10.109628183187));
#84372=CARTESIAN_POINT('Ctrl Pts',(16.6477625455389,-18.5923573635147,-10.1087745113515));
#84373=CARTESIAN_POINT('Ctrl Pts',(16.6466902780684,-18.5986338039992,-10.1083934713747));
#84374=CARTESIAN_POINT('Ctrl Pts',(16.6446635347929,-18.6108283881455,-10.1076554498014));
#84375=CARTESIAN_POINT('Ctrl Pts',(16.6437058477124,-18.6167459297388,-10.1072983696492));
#84376=CARTESIAN_POINT('Ctrl Pts',(16.6416603183947,-18.6297348257842,-10.1065168546868));
#84377=CARTESIAN_POINT('Ctrl Pts',(16.6405831593277,-18.6368078065209,-10.1060927609098));
#84378=CARTESIAN_POINT('Ctrl Pts',(16.6380227876596,-18.654212385253,-10.1050527299054));
#84379=CARTESIAN_POINT('Ctrl Pts',(16.6365800759984,-18.6645498193423,-10.1044380685977));
#84380=CARTESIAN_POINT('Ctrl Pts',(16.6230153914468,-18.7672893702876,-10.0983585237394));
#84381=CARTESIAN_POINT('Ctrl Pts',(16.6169303822883,-18.8603894548246,-10.0930911632084));
#84382=CARTESIAN_POINT('Ctrl Pts',(16.617000600774,-18.9535948907958,-10.0879364327122));
#84383=CARTESIAN_POINT('Ctrl Pts',(16.617000598892,-18.9535923908226,-10.0879365709734));
#84384=CARTESIAN_POINT('Ctrl Pts',(16.6171096392611,-19.0985557959938,-10.0799193607352));
#84385=CARTESIAN_POINT('Ctrl Pts',(16.6321076022928,-19.2431231720195,-10.0722250138809));
#84386=CARTESIAN_POINT('Ctrl Pts',(16.6753573988837,-19.4500950284509,-10.0604951744654));
#84387=CARTESIAN_POINT('Ctrl Pts',(16.6920108411014,-19.5144825012199,-10.056735958022));
#84388=CARTESIAN_POINT('Ctrl Pts',(16.7155915269103,-19.5906648131193,-10.0520405658893));
#84389=CARTESIAN_POINT('Ctrl Pts',(16.7196392101853,-19.6033187361381,-10.0512522809237));
#84390=CARTESIAN_POINT('Ctrl Pts',(16.7254517172716,-19.6209172932602,-10.0501431585338));
#84391=CARTESIAN_POINT('Ctrl Pts',(16.7271163361503,-19.6258950272122,-10.0498280068219));
#84392=CARTESIAN_POINT('Ctrl Pts',(16.7299779737093,-19.6343475839671,-10.0492903272845));
#84393=CARTESIAN_POINT('Ctrl Pts',(16.7311655755179,-19.6378256156405,-10.0490683541719));
#84394=CARTESIAN_POINT('Ctrl Pts',(16.7334553551712,-19.6444748336374,-10.0486425620907));
#84395=CARTESIAN_POINT('Ctrl Pts',(16.7345560270915,-19.6476465122525,-10.0484388371499));
#84396=CARTESIAN_POINT('Ctrl Pts',(16.7374836519418,-19.6560183603001,-10.0478994731463));
#84397=CARTESIAN_POINT('Ctrl Pts',(16.7393233626526,-19.6612139948961,-10.0475630863369));
#84398=CARTESIAN_POINT('Ctrl Pts',(16.7425839020076,-19.6703092302424,-10.0469713956746));
#84399=CARTESIAN_POINT('Ctrl Pts',(16.743995952389,-19.6742119599656,-10.0467165876099));
#84400=CARTESIAN_POINT('Ctrl Pts',(16.7454194499602,-19.6781104571642,-10.0464611570501));
#84401=CARTESIAN_POINT('Origin',(18.734,-18.952,0.));
#84402=CARTESIAN_POINT('',(16.7454193049359,-19.6781100599899,-9.24346979696294));
#84403=CARTESIAN_POINT('',(16.7454194499637,-19.6781104571739,-9.46634969428706));
#84404=CARTESIAN_POINT('',(16.7454194499637,-19.6781104571739,0.));
#84405=CARTESIAN_POINT('',(16.6163914686439,-18.9501065431989,-9.51094371951101));
#84406=CARTESIAN_POINT('Ctrl Pts',(16.7454194499637,-19.6781104571739,-9.46634969428706));
#84407=CARTESIAN_POINT('Ctrl Pts',(16.720738363517,-19.6105169829623,-9.47066127906487));
#84408=CARTESIAN_POINT('Ctrl Pts',(16.6995057447712,-19.5416582823502,-9.47497286384268));
#84409=CARTESIAN_POINT('Ctrl Pts',(16.6818386273343,-19.4719256682822,-9.4792844486205));
#84410=CARTESIAN_POINT('Ctrl Pts',(16.6641689582128,-19.4021829826427,-9.48359665612607));
#84411=CARTESIAN_POINT('Ctrl Pts',(16.6500659224548,-19.3315666185462,-9.48790886363164));
#84412=CARTESIAN_POINT('Ctrl Pts',(16.6395956396387,-19.2604791326809,-9.49222107113721));
#84413=CARTESIAN_POINT('Ctrl Pts',(16.6291143284222,-19.1893167700171,-9.49653782071216));
#84414=CARTESIAN_POINT('Ctrl Pts',(16.6222734602416,-19.1176827900521,-9.5008545702871));
#84415=CARTESIAN_POINT('Ctrl Pts',(16.6190872658347,-19.045984716126,-9.50517131986205));
#84416=CARTESIAN_POINT('Ctrl Pts',(16.6176670680628,-19.0140263884681,-9.50709544543166));
#84417=CARTESIAN_POINT('Ctrl Pts',(16.6169722855429,-18.9820553302898,-9.50901957100126));
#84418=CARTESIAN_POINT('Ctrl Pts',(16.6170008459316,-18.9501074689745,-9.51094369657087));
#84419=CARTESIAN_POINT('Ctrl Pts',(16.6163525130807,-18.950106484017,-9.51094372097751));
#84420=CARTESIAN_POINT('Ctrl Pts',(16.6150298054201,-18.8071177642836,-9.51955279572482));
#84421=CARTESIAN_POINT('Ctrl Pts',(16.6934794852886,-17.9614815818345,-9.57055380603263));
#84422=CARTESIAN_POINT('Ctrl Pts',(17.8308508267527,-16.6173368175504,-9.66394675190085));
#84423=CARTESIAN_POINT('Ctrl Pts',(20.2082247500812,-16.9288855714837,-9.79112255858234));
#84424=CARTESIAN_POINT('Ctrl Pts',(21.2330889659179,-19.0965162449378,-9.91829836526374));
#84425=CARTESIAN_POINT('Ctrl Pts',(19.9651941664791,-21.1315622333511,-10.0454741719452));
#84426=CARTESIAN_POINT('Ctrl Pts',(17.7787242232772,-21.1638771367373,-10.1614588019006));
#84427=CARTESIAN_POINT('Ctrl Pts',(16.9288259160256,-20.1636739641463,-10.2350514962957));
#84428=CARTESIAN_POINT('Ctrl Pts',(16.7460269997163,-19.6778790908883,-10.2662522551303));
#84429=CARTESIAN_POINT('Ctrl Pts',(16.7454194499602,-19.6781104571642,-10.0464611570501));
#84430=CARTESIAN_POINT('Ctrl Pts',(16.7487705800937,-19.6872881134538,-10.0458598346008));
#84431=CARTESIAN_POINT('Ctrl Pts',(16.7521851509511,-19.6964423129619,-10.0452550625254));
#84432=CARTESIAN_POINT('Ctrl Pts',(16.8148899433013,-19.8610598294149,-10.0342936653091));
#84433=CARTESIAN_POINT('Ctrl Pts',(16.8922364625482,-20.0090121106089,-10.0231059329381));
#84434=CARTESIAN_POINT('Ctrl Pts',(17.0314061086661,-20.2126792326606,-10.0069007354659));
#84435=CARTESIAN_POINT('Ctrl Pts',(17.0804528128878,-20.2763571406402,-10.0016885341233));
#84436=CARTESIAN_POINT('Ctrl Pts',(17.1587312159261,-20.3668369246799,-9.99410804453697));
#84437=CARTESIAN_POINT('Ctrl Pts',(17.1852837348339,-20.3958537006746,-9.99164686094173));
#84438=CARTESIAN_POINT('Ctrl Pts',(17.2310837946067,-20.4431861352719,-9.98758039807538));
#84439=CARTESIAN_POINT('Ctrl Pts',(17.2498945865422,-20.4619087497938,-9.98595738198995));
#84440=CARTESIAN_POINT('Ctrl Pts',(17.2761201267121,-20.4870475910786,-9.98375697301453));
#84441=CARTESIAN_POINT('Ctrl Pts',(17.2832341192949,-20.4937727446786,-9.98316616620807));
#84442=CARTESIAN_POINT('Ctrl Pts',(17.2947526968862,-20.5045114175436,-9.98221919500483));
#84443=CARTESIAN_POINT('Ctrl Pts',(17.2991279619979,-20.5085560500066,-9.9818616964551));
#84444=CARTESIAN_POINT('Ctrl Pts',(17.308279409707,-20.5169445606849,-9.98111848350948));
#84445=CARTESIAN_POINT('Ctrl Pts',(17.3130585100684,-20.5212851758742,-9.98073291007807));
#84446=CARTESIAN_POINT('Ctrl Pts',(17.3241384488046,-20.5312564099933,-9.97984480770873));
#84447=CARTESIAN_POINT('Ctrl Pts',(17.3304533192749,-20.5368713260791,-9.97934294330554));
#84448=CARTESIAN_POINT('Ctrl Pts',(17.3475251730836,-20.551868836075,-9.97799754901092));
#84449=CARTESIAN_POINT('Ctrl Pts',(17.358343826291,-20.5611807993244,-9.97715695212527));
#84450=CARTESIAN_POINT('Ctrl Pts',(17.4588253890171,-20.6459145261259,-9.96945662525717));
#84451=CARTESIAN_POINT('Ctrl Pts',(17.5545157297192,-20.7138850312153,-9.96291554066431));
#84452=CARTESIAN_POINT('Ctrl Pts',(17.7962403809785,-20.8570211747457,-9.94753795322736));
#84453=CARTESIAN_POINT('Ctrl Pts',(17.9463144762433,-20.9238108435326,-9.93888737341477));
#84454=CARTESIAN_POINT('Ctrl Pts',(18.1324876106429,-20.9819888684044,-9.92767339637413));
#84455=CARTESIAN_POINT('Ctrl Pts',(18.1626149728676,-20.9906738030423,-9.92584312774557));
#84456=CARTESIAN_POINT('Ctrl Pts',(18.1998433757607,-21.0005157923087,-9.92354994607645));
#84457=CARTESIAN_POINT('Ctrl Pts',(18.2067736724179,-21.0023103781449,-9.92312172551355));
#84458=CARTESIAN_POINT('Ctrl Pts',(18.2176792610823,-21.0050754098504,-9.92244559294023));
#84459=CARTESIAN_POINT('Ctrl Pts',(18.2216485659944,-21.0060695585567,-9.92219902767828));
#84460=CARTESIAN_POINT('Ctrl Pts',(18.2290907245816,-21.0079106015636,-9.9217358066966));
#84461=CARTESIAN_POINT('Ctrl Pts',(18.2325628494293,-21.0087602099854,-9.92151930971906));
#84462=CARTESIAN_POINT('Ctrl Pts',(18.2405165857451,-21.0106851048478,-9.92102250717175));
#84463=CARTESIAN_POINT('Ctrl Pts',(18.2449995541821,-21.0117545494863,-9.92074187039057));
#84464=CARTESIAN_POINT('Ctrl Pts',(18.2588699155176,-21.0150155912093,-9.91987172683355));
#84465=CARTESIAN_POINT('Ctrl Pts',(18.268268658918,-21.0171576783912,-9.91927949039792));
#84466=CARTESIAN_POINT('Ctrl Pts',(18.3638848060111,-21.0382638455474,-9.91323026294764));
#84467=CARTESIAN_POINT('Ctrl Pts',(18.4511844512886,-21.0518794793575,-9.90751051502923));
#84468=CARTESIAN_POINT('Ctrl Pts',(18.6668380104197,-21.07182149918,-9.89328340561099));
#84469=CARTESIAN_POINT('Ctrl Pts',(18.795428898532,-21.0719963152216,-9.88473130295712));
#84470=CARTESIAN_POINT('Ctrl Pts',(18.9852673388954,-21.0549577562344,-9.87241271069616));
#84471=CARTESIAN_POINT('Ctrl Pts',(19.0470167231885,-21.0466570805686,-9.86845064721064));
#84472=CARTESIAN_POINT('Ctrl Pts',(19.1451810672345,-21.0290224095671,-9.86223503603126));
#84473=CARTESIAN_POINT('Ctrl Pts',(19.1818664647965,-21.0214221103261,-9.85993072719303));
#84474=CARTESIAN_POINT('Ctrl Pts',(19.229192757228,-21.0102996832341,-9.85698030549256));
#84475=CARTESIAN_POINT('Ctrl Pts',(19.2400325336125,-21.0076615809032,-9.85630604686218));
#84476=CARTESIAN_POINT('Ctrl Pts',(19.2576146247104,-21.0032350838827,-9.85521474389727));
#84477=CARTESIAN_POINT('Ctrl Pts',(19.2643697398668,-21.0014988620166,-9.85479602480717));
#84478=CARTESIAN_POINT('Ctrl Pts',(19.2773351036564,-20.9980980671859,-9.85399340316984));
#84479=CARTESIAN_POINT('Ctrl Pts',(19.2835465814626,-20.9964385272289,-9.85360934285446));
#84480=CARTESIAN_POINT('Ctrl Pts',(19.2977391837189,-20.9925772899423,-9.85273281632792));
#84481=CARTESIAN_POINT('Ctrl Pts',(19.305715177932,-20.9903570103843,-9.85224095883366));
#84482=CARTESIAN_POINT('Ctrl Pts',(19.3268436071897,-20.984341713223,-9.85093985787687));
#84483=CARTESIAN_POINT('Ctrl Pts',(19.3399727434232,-20.9804657821252,-9.85013324939695));
#84484=CARTESIAN_POINT('Ctrl Pts',(19.4381168812101,-20.9504541337861,-9.84411603218965));
#84485=CARTESIAN_POINT('Ctrl Pts',(19.5214522269294,-20.9191098740275,-9.83908225683098));
#84486=CARTESIAN_POINT('Ctrl Pts',(19.7313864581444,-20.8246610824248,-9.82633015447441));
#84487=CARTESIAN_POINT('Ctrl Pts',(19.8540672755892,-20.7539674384573,-9.81882079775667));
#84488=CARTESIAN_POINT('Ctrl Pts',(20.0134925739095,-20.6394881366564,-9.80797731963053));
#84489=CARTESIAN_POINT('Ctrl Pts',(20.0569216447132,-20.6056610715429,-9.80489312583969));
#84490=CARTESIAN_POINT('Ctrl Pts',(20.1206848305545,-20.5518751353147,-9.8000808919658));
#84491=CARTESIAN_POINT('Ctrl Pts',(20.1420174350213,-20.5331331355077,-9.79841933814992));
#84492=CARTESIAN_POINT('Ctrl Pts',(20.168083384129,-20.5092867310699,-9.79631441044709));
#84493=CARTESIAN_POINT('Ctrl Pts',(20.173178181235,-20.5045795551338,-9.79589933593127));
#84494=CARTESIAN_POINT('Ctrl Pts',(20.1812055337909,-20.4970894753331,-9.79523936709984));
#84495=CARTESIAN_POINT('Ctrl Pts',(20.1841534605497,-20.4943230154693,-9.79499571437365));
#84496=CARTESIAN_POINT('Ctrl Pts',(20.1896996377925,-20.4890882888963,-9.79453483107102));
#84497=CARTESIAN_POINT('Ctrl Pts',(20.1922995514029,-20.4866218625421,-9.79431774053349));
#84498=CARTESIAN_POINT('Ctrl Pts',(20.1982311387073,-20.4809661357236,-9.79382008819772));
#84499=CARTESIAN_POINT('Ctrl Pts',(20.2015586570383,-20.4777725449662,-9.79353919610343));
#84500=CARTESIAN_POINT('Ctrl Pts',(20.2103686539848,-20.4692616548018,-9.79279099112213));
#84501=CARTESIAN_POINT('Ctrl Pts',(20.2158327804624,-20.4639255730068,-9.79232226894043));
#84502=CARTESIAN_POINT('Ctrl Pts',(20.2539995434603,-20.4262475560296,-9.78901607269487));
#84503=CARTESIAN_POINT('Ctrl Pts',(20.2856669391502,-20.392879412843,-9.7861059525481));
#84504=CARTESIAN_POINT('Ctrl Pts',(20.4208039546154,-20.2408601972975,-9.77302745189414));
#84505=CARTESIAN_POINT('Ctrl Pts',(20.5119397262914,-20.111914263051,-9.76243943244153));
#84506=CARTESIAN_POINT('Ctrl Pts',(20.6351493005773,-19.8884198288713,-9.74583522376284));
#84507=CARTESIAN_POINT('Ctrl Pts',(20.6763731026431,-19.7996096085827,-9.73961548559119));
#84508=CARTESIAN_POINT('Ctrl Pts',(20.7190560586598,-19.6880103771488,-9.73227405897855));
#84509=CARTESIAN_POINT('Ctrl Pts',(20.7264880543991,-19.6676467279378,-9.73095259784948));
#84510=CARTESIAN_POINT('Ctrl Pts',(20.7365804918525,-19.6386166417251,-9.72909370309057));
#84511=CARTESIAN_POINT('Ctrl Pts',(20.7394998699028,-19.6300422662695,-9.72854771052524));
#84512=CARTESIAN_POINT('Ctrl Pts',(20.7444307264143,-19.6152495772273,-9.72761092211941));
#84513=CARTESIAN_POINT('Ctrl Pts',(20.7464685874899,-19.6090402523865,-9.72721925879928));
#84514=CARTESIAN_POINT('Ctrl Pts',(20.7503084077861,-19.5971549169186,-9.72647251146765));
#84515=CARTESIAN_POINT('Ctrl Pts',(20.7521152305639,-19.5914805543681,-9.7261172703924));
#84516=CARTESIAN_POINT('Ctrl Pts',(20.756736511254,-19.5767526642914,-9.72519849665849));
#84517=CARTESIAN_POINT('Ctrl Pts',(20.7595141571454,-19.5676876555111,-9.72463617547587));
#84518=CARTESIAN_POINT('Ctrl Pts',(20.7687051334847,-19.536956871973,-9.72274038793743));
#84519=CARTESIAN_POINT('Ctrl Pts',(20.7748326166676,-19.5152067213116,-9.72141623835557));
#84520=CARTESIAN_POINT('Ctrl Pts',(20.8267419806815,-19.3189641531164,-9.70961601923621));
#84521=CARTESIAN_POINT('Ctrl Pts',(20.8503939628842,-19.1393891766988,-9.69994105044149));
#84522=CARTESIAN_POINT('Ctrl Pts',(20.8512640462748,-18.8753638286044,-9.68556286600716));
#84523=CARTESIAN_POINT('Ctrl Pts',(20.8465857594597,-18.7918146282843,-9.68097533658553));
#84524=CARTESIAN_POINT('Ctrl Pts',(20.83273510524,-18.6720618887445,-9.67408633509576));
#84525=CARTESIAN_POINT('Ctrl Pts',(20.8275295954145,-18.6354753608906,-9.67193852902863));
#84526=CARTESIAN_POINT('Ctrl Pts',(20.8201158532339,-18.5916304462376,-9.66929255327628));
#84527=CARTESIAN_POINT('Ctrl Pts',(20.8188224028559,-18.58422138032,-9.66884293404462));
#84528=CARTESIAN_POINT('Ctrl Pts',(20.8167502737151,-18.5727142277777,-9.66814052339554));
#84529=CARTESIAN_POINT('Ctrl Pts',(20.815998901674,-18.5686111994208,-9.66788925769288));
#84530=CARTESIAN_POINT('Ctrl Pts',(20.8145829340087,-18.561005930782,-9.66742196685207));
#84531=CARTESIAN_POINT('Ctrl Pts',(20.8139216170854,-18.557503138619,-9.66720612963331));
#84532=CARTESIAN_POINT('Ctrl Pts',(20.8124064858603,-18.5495876740574,-9.66671700346674));
#84533=CARTESIAN_POINT('Ctrl Pts',(20.8115474688085,-18.5451760644671,-9.6664434225099));
#84534=CARTESIAN_POINT('Ctrl Pts',(20.8089703108162,-18.5321617353532,-9.6656335535975));
#84535=CARTESIAN_POINT('Ctrl Pts',(20.8072127619355,-18.5235670450785,-9.66509509832949));
#84536=CARTESIAN_POINT('Ctrl Pts',(20.7941088895004,-18.4614563504302,-9.66117891153828));
#84537=CARTESIAN_POINT('Ctrl Pts',(20.7807463196187,-18.4083915891833,-9.65769912493189));
#84538=CARTESIAN_POINT('Ctrl Pts',(20.7569451113049,-18.3272823588542,-9.65223131095082));
#84539=CARTESIAN_POINT('Ctrl Pts',(20.7479407525649,-18.2988372357528,-9.65028466107274));
#84540=CARTESIAN_POINT('Ctrl Pts',(20.6966405512842,-18.147939258153,-9.63983111712647));
#84541=CARTESIAN_POINT('Ctrl Pts',(20.6437683453331,-18.0293624064292,-9.63118798340045));
#84542=CARTESIAN_POINT('Ctrl Pts',(20.5373132122674,-17.8395688736772,-9.61709965361327));
#84543=CARTESIAN_POINT('Ctrl Pts',(20.4894868974471,-17.7655301540048,-9.61152494773811));
#84544=CARTESIAN_POINT('Ctrl Pts',(20.425008091196,-17.6781865198193,-9.60486235783854));
#84545=CARTESIAN_POINT('Ctrl Pts',(20.4125951025672,-17.6618730005151,-9.60361371622558));
#84546=CARTESIAN_POINT('Ctrl Pts',(20.3944819989994,-17.6387723084949,-9.60183889997603));
#84547=CARTESIAN_POINT('Ctrl Pts',(20.3889734634666,-17.6318370260897,-9.60130518176159));
#84548=CARTESIAN_POINT('Ctrl Pts',(20.3793475157917,-17.619872832764,-9.60038284195804));
#84549=CARTESIAN_POINT('Ctrl Pts',(20.375250199588,-17.6148279762034,-9.59999342221179));
#84550=CARTESIAN_POINT('Ctrl Pts',(20.3673267025798,-17.6051633869561,-9.59924639093293));
#84551=CARTESIAN_POINT('Ctrl Pts',(20.3635039969832,-17.6005408979361,-9.59888864427572));
#84552=CARTESIAN_POINT('Ctrl Pts',(20.3534366718736,-17.5884721101804,-9.59795338779382));
#84553=CARTESIAN_POINT('Ctrl Pts',(20.347160289299,-17.5810523983983,-9.59737717893864));
#84554=CARTESIAN_POINT('Ctrl Pts',(20.3251920539414,-17.5554421017974,-9.59538374936086));
#84555=CARTESIAN_POINT('Ctrl Pts',(20.3092414694154,-17.537475168864,-9.59397721905543));
#84556=CARTESIAN_POINT('Ctrl Pts',(20.1932899243854,-17.4112603013938,-9.58402816140778));
#84557=CARTESIAN_POINT('Ctrl Pts',(20.0825309530204,-17.3134406247597,-9.57598921309175));
#84558=CARTESIAN_POINT('Ctrl Pts',(19.924281372916,-17.2006801613959,-9.56543632537456));
#84559=CARTESIAN_POINT('Ctrl Pts',(19.8851714750098,-17.1747281987349,-9.5628909327256));
#84560=CARTESIAN_POINT('Ctrl Pts',(19.7844797586393,-17.1126316795459,-9.55641959030261));
#84561=CARTESIAN_POINT('Ctrl Pts',(19.7218759288467,-17.0782649224539,-9.55247019126166));
#84562=CARTESIAN_POINT('Ctrl Pts',(19.6274567465628,-17.0324815993257,-9.54645205774746));
#84563=CARTESIAN_POINT('Ctrl Pts',(19.5969096306861,-17.0185568195946,-9.54449579895512));
#84564=CARTESIAN_POINT('Ctrl Pts',(19.5593239837972,-17.0024916597132,-9.54206244678197));
#84565=CARTESIAN_POINT('Ctrl Pts',(19.5525868360795,-16.9996531979863,-9.54162525725391));
#84566=CARTESIAN_POINT('Ctrl Pts',(19.5420253048286,-16.9952677431455,-9.5409381048969));
#84567=CARTESIAN_POINT('Ctrl Pts',(19.5382107975635,-16.9936969053098,-9.54068956264767));
#84568=CARTESIAN_POINT('Ctrl Pts',(19.5310869187825,-16.9907875720626,-9.54022467057551));
#84569=CARTESIAN_POINT('Ctrl Pts',(19.5277787447478,-16.9894462944071,-9.54000849190005));
#84570=CARTESIAN_POINT('Ctrl Pts',(19.5202385190781,-16.9864113426655,-9.53951510361877));
#84571=CARTESIAN_POINT('Ctrl Pts',(19.5160043967038,-16.9847229728984,-9.53923758006645));
#84572=CARTESIAN_POINT('Ctrl Pts',(19.5049816460905,-16.9803688241527,-9.53851394819959));
#84573=CARTESIAN_POINT('Ctrl Pts',(19.4981847022136,-16.9777244545004,-9.53806660435822));
#84574=CARTESIAN_POINT('Ctrl Pts',(19.4548181590024,-16.9611100777212,-9.53520584775666));
#84575=CARTESIAN_POINT('Ctrl Pts',(19.4178831164481,-16.9481225246284,-9.53273978951299));
#84576=CARTESIAN_POINT('Ctrl Pts',(19.3688624524125,-16.9323983247203,-9.52944737596279));
#84577=CARTESIAN_POINT('Ctrl Pts',(19.3570802245899,-16.928732275929,-9.52865457279627));
#84578=CARTESIAN_POINT('Ctrl Pts',(19.3221509476063,-16.9181980410258,-9.52630119208308));
#84579=CARTESIAN_POINT('Ctrl Pts',(19.2989180870275,-16.9116227215546,-9.52473193113092));
#84580=CARTESIAN_POINT('Ctrl Pts',(19.136220013105,-16.8685680083954,-9.51373620452499));
#84581=CARTESIAN_POINT('Ctrl Pts',(18.9934449950039,-16.8460172980108,-9.50408906827816));
#84582=CARTESIAN_POINT('Ctrl Pts',(18.7877688399188,-16.8347805082826,-9.49078080342547));
#84583=CARTESIAN_POINT('Ctrl Pts',(18.7259288399144,-16.8341129748524,-9.48684921219987));
#84584=CARTESIAN_POINT('Ctrl Pts',(18.6269048133701,-16.8373823397465,-9.48067558989718));
#84585=CARTESIAN_POINT('Ctrl Pts',(18.5897034138333,-16.8395947358536,-9.47838364300904));
#84586=CARTESIAN_POINT('Ctrl Pts',(18.5414838612195,-16.8437423014528,-9.47544654793898));
#84587=CARTESIAN_POINT('Ctrl Pts',(18.5303974114124,-16.8447840688444,-9.47477356748234));
#84588=CARTESIAN_POINT('Ctrl Pts',(18.5123855101946,-16.8466200822429,-9.47368381678425));
#84589=CARTESIAN_POINT('Ctrl Pts',(18.5054549613242,-16.8473611361349,-9.47326538066321));
#84590=CARTESIAN_POINT('Ctrl Pts',(18.4921372994333,-16.8488516960358,-9.47246295685561));
#84591=CARTESIAN_POINT('Ctrl Pts',(18.4857497040793,-16.8495961029391,-9.47207881325076));
#84592=CARTESIAN_POINT('Ctrl Pts',(18.4711367175062,-16.8513666187687,-9.47120162003065));
#84593=CARTESIAN_POINT('Ctrl Pts',(18.4629137290526,-16.8524119584277,-9.47070918235473));
#84594=CARTESIAN_POINT('Ctrl Pts',(18.4410945244786,-16.8553160258346,-9.46940552674511));
#84595=CARTESIAN_POINT('Ctrl Pts',(18.4275097403157,-16.8572587178701,-9.46859696055655));
#84596=CARTESIAN_POINT('Ctrl Pts',(18.3247121567189,-16.8729807280252,-9.46250012681056));
#84597=CARTESIAN_POINT('Ctrl Pts',(18.2364381115432,-16.8923221844788,-9.45739434800246));
#84598=CARTESIAN_POINT('Ctrl Pts',(18.0155894357492,-16.9557453733172,-9.44467437709994));
#84599=CARTESIAN_POINT('Ctrl Pts',(17.8856587127161,-17.0074019747641,-9.43725491486124));
#84600=CARTESIAN_POINT('Ctrl Pts',(17.712639698633,-17.0968532881045,-9.42649617652613));
#84601=CARTESIAN_POINT('Ctrl Pts',(17.664540704521,-17.1241591554437,-9.42339806776635));
#84602=CARTESIAN_POINT('Ctrl Pts',(17.5933680507303,-17.1683354879316,-9.41856617912751));
#84603=CARTESIAN_POINT('Ctrl Pts',(17.5694739384615,-17.1838429913178,-9.41689953252225));
#84604=CARTESIAN_POINT('Ctrl Pts',(17.5401543141684,-17.2037237941696,-9.41478891120607));
#84605=CARTESIAN_POINT('Ctrl Pts',(17.5344266243528,-17.2076488521969,-9.41437341909254));
#84606=CARTESIAN_POINT('Ctrl Pts',(17.5253935827557,-17.2139045237138,-9.41371293663021));
#84607=CARTESIAN_POINT('Ctrl Pts',(17.5220753642248,-17.2162165938512,-9.41346919115557));
#84608=CARTESIAN_POINT('Ctrl Pts',(17.5158296069448,-17.2205951558227,-9.41300823591552));
#84609=CARTESIAN_POINT('Ctrl Pts',(17.5129006825669,-17.2226595774096,-9.41279116679348));
#84610=CARTESIAN_POINT('Ctrl Pts',(17.5062161343094,-17.2273965596402,-9.41229369831953));
#84611=CARTESIAN_POINT('Ctrl Pts',(17.5024639929694,-17.2300739534431,-9.41201296955642));
#84612=CARTESIAN_POINT('Ctrl Pts',(17.4925254610199,-17.2372148345733,-9.41126548164981));
#84613=CARTESIAN_POINT('Ctrl Pts',(17.4863544670865,-17.2416994957955,-9.41079731741055));
#84614=CARTESIAN_POINT('Ctrl Pts',(17.4432975305892,-17.2733473988742,-9.40750318604318));
#84615=CARTESIAN_POINT('Ctrl Pts',(17.4072803261857,-17.3016662039632,-9.40460515528195));
#84616=CARTESIAN_POINT('Ctrl Pts',(17.3434297880869,-17.3553106914298,-9.39924370613024));
#84617=CARTESIAN_POINT('Ctrl Pts',(17.3152969373005,-17.3802545828514,-9.39679632781525));
#84618=CARTESIAN_POINT('Ctrl Pts',(17.192180394829,-17.4954149916012,-9.38574620355505));
#84619=CARTESIAN_POINT('Ctrl Pts',(17.1050205672822,-17.5935901668398,-9.37700301427132));
#84620=CARTESIAN_POINT('Ctrl Pts',(16.9752026480569,-17.7704210816275,-9.36279856028141));
#84621=CARTESIAN_POINT('Ctrl Pts',(16.9274171300745,-17.8448601604884,-9.35720316407805));
#84622=CARTESIAN_POINT('Ctrl Pts',(16.8744284015705,-17.9400196549519,-9.35051865954794));
#84623=CARTESIAN_POINT('Ctrl Pts',(16.8646987124888,-17.958106901319,-9.34926760661699));
#84624=CARTESIAN_POINT('Ctrl Pts',(16.8511486069233,-17.9841993022664,-9.34748999740643));
#84625=CARTESIAN_POINT('Ctrl Pts',(16.8471131270219,-17.992090894271,-9.34695586490234));
#84626=CARTESIAN_POINT('Ctrl Pts',(16.8402042019512,-18.0058135870329,-9.34603303937244));
#84627=CARTESIAN_POINT('Ctrl Pts',(16.837307855725,-18.0116329630942,-9.34564354586782));
#84628=CARTESIAN_POINT('Ctrl Pts',(16.8317911214945,-18.0228464371983,-9.34489653270058));
#84629=CARTESIAN_POINT('Ctrl Pts',(16.829166763936,-18.0282385022869,-9.34453887715261));
#84630=CARTESIAN_POINT('Ctrl Pts',(16.8223533123695,-18.0423900742458,-9.34360421261495));
#84631=CARTESIAN_POINT('Ctrl Pts',(16.8182014766042,-18.0511674418156,-9.34302850135214));
#84632=CARTESIAN_POINT('Ctrl Pts',(16.8040088680704,-18.0817138836066,-9.34103852658906));
#84633=CARTESIAN_POINT('Ctrl Pts',(16.7942773423429,-18.1036252160942,-9.33963490353653));
#84634=CARTESIAN_POINT('Ctrl Pts',(16.7250855536645,-18.2668346877018,-9.3293440439758));
#84635=CARTESIAN_POINT('Ctrl Pts',(16.6807559356853,-18.4140553695192,-9.32100721039236));
#84636=CARTESIAN_POINT('Ctrl Pts',(16.6289120188436,-18.6927191509291,-9.30561469461767));
#84637=CARTESIAN_POINT('Ctrl Pts',(16.6169601914202,-18.8225565402336,-9.29857228728212));
#84638=CARTESIAN_POINT('Ctrl Pts',(16.6170011042386,-18.9559243141497,-9.29078130781142));
#84639=CARTESIAN_POINT('Ctrl Pts',(16.6170097079818,-18.9591991753601,-9.2905896487255));
#84640=CARTESIAN_POINT('Ctrl Pts',(16.6171033846654,-18.9781328626562,-9.28947947249069));
#84641=CARTESIAN_POINT('Ctrl Pts',(16.617354592849,-18.9937898859883,-9.28855313985671));
#84642=CARTESIAN_POINT('Ctrl Pts',(16.6179364383181,-19.015225593477,-9.28727182670056));
#84643=CARTESIAN_POINT('Ctrl Pts',(16.6181171280115,-19.0210082820074,-9.28692486276551));
#84644=CARTESIAN_POINT('Ctrl Pts',(16.618441992775,-19.0301981290071,-9.28637129038767));
#84645=CARTESIAN_POINT('Ctrl Pts',(16.6185707023212,-19.0336058543001,-9.28616554187761));
#84646=CARTESIAN_POINT('Ctrl Pts',(16.6188536012539,-19.0406449231496,-9.28573953272618));
#84647=CARTESIAN_POINT('Ctrl Pts',(16.6190089084551,-19.0442761748026,-9.28551920786138));
#84648=CARTESIAN_POINT('Ctrl Pts',(16.6194013860905,-19.0529306252594,-9.28499279386702));
#84649=CARTESIAN_POINT('Ctrl Pts',(16.6196471048459,-19.0579533983379,-9.28468622986837));
#84650=CARTESIAN_POINT('Ctrl Pts',(16.6205368676228,-19.0749034750163,-9.28364825052643));
#84651=CARTESIAN_POINT('Ctrl Pts',(16.6212639473949,-19.0868259360013,-9.28291240768569));
#84652=CARTESIAN_POINT('Ctrl Pts',(16.631113687836,-19.2285839076868,-9.27409998991241));
#84653=CARTESIAN_POINT('Ctrl Pts',(16.6520896332326,-19.3573045948984,-9.265483365158));
#84654=CARTESIAN_POINT('Ctrl Pts',(16.701839122724,-19.5492021999487,-9.25238340889672));
#84655=CARTESIAN_POINT('Ctrl Pts',(16.7220914885675,-19.6142227130923,-9.24789463062267));
#84656=CARTESIAN_POINT('Ctrl Pts',(16.7454193049359,-19.6781100599899,-9.24346979696294));
#84657=CARTESIAN_POINT('Origin',(18.734,-18.952,0.));
#84658=CARTESIAN_POINT('',(16.7454194499637,-19.6781104571739,-8.4444886490522));
#84659=CARTESIAN_POINT('',(16.7454194712032,-19.678110515342,-8.66553666923996));
#84660=CARTESIAN_POINT('',(16.7454194499637,-19.6781104571739,0.));
#84661=CARTESIAN_POINT('',(16.6170000013281,-18.9519250126714,-8.71094372102528));
#84662=CARTESIAN_POINT('Ctrl Pts',(16.7454194712032,-19.678110515342,-8.66553666923996));
#84663=CARTESIAN_POINT('Ctrl Pts',(16.6904356127053,-19.527527610816,-8.67608242901258));
#84664=CARTESIAN_POINT('Ctrl Pts',(16.6527074043694,-19.3711105565511,-8.68676264432225));
#84665=CARTESIAN_POINT('Ctrl Pts',(16.6297591054065,-19.1855832829213,-8.69860360219042));
#84666=CARTESIAN_POINT('Ctrl Pts',(16.6270006245378,-19.1592308344624,-8.70026804571858));
#84667=CARTESIAN_POINT('Ctrl Pts',(16.6216845085739,-19.0972227551114,-8.70414333167712));
#84668=CARTESIAN_POINT('Ctrl Pts',(16.6195337123929,-19.0615397043015,-8.70634146733557));
#84669=CARTESIAN_POINT('Ctrl Pts',(16.617898153749,-19.0146623185697,-8.70918909189148));
#84670=CARTESIAN_POINT('Ctrl Pts',(16.6175971721877,-19.0035040559628,-8.70986395115042));
#84671=CARTESIAN_POINT('Ctrl Pts',(16.6172522425384,-18.9854074934492,-8.71095376412891));
#84672=CARTESIAN_POINT('Ctrl Pts',(16.6171541291233,-18.9784705510505,-8.71137040718873));
#84673=CARTESIAN_POINT('Ctrl Pts',(16.6170502016031,-18.967207401971,-8.71204511525387));
#84674=CARTESIAN_POINT('Ctrl Pts',(16.6170235457565,-18.9628814804057,-8.71230383078575));
#84675=CARTESIAN_POINT('Ctrl Pts',(16.617003429385,-18.9563852150012,-8.71269171670242));
#84676=CARTESIAN_POINT('Ctrl Pts',(16.6170000462402,-18.9542149335066,-8.71282119677421));
#84677=CARTESIAN_POINT('Ctrl Pts',(16.6170000004708,-18.9520446456796,-8.71295057259137));
#84678=CARTESIAN_POINT('Ctrl Pts',(16.6170000013281,-18.9519250126714,-8.71094372102528));
#84679=CARTESIAN_POINT('Ctrl Pts',(16.6170027209272,-18.8751468230115,-8.71553605185447));
#84680=CARTESIAN_POINT('Ctrl Pts',(16.6211865549027,-18.7984540523296,-8.72012838268367));
#84681=CARTESIAN_POINT('Ctrl Pts',(16.6294980530145,-18.7223033410468,-8.72472071351286));
#84682=CARTESIAN_POINT('Ctrl Pts',(16.637833810921,-18.6459303592898,-8.7293264485445));
#84683=CARTESIAN_POINT('Ctrl Pts',(16.6503212662752,-18.570103004567,-8.73393218357614));
#84684=CARTESIAN_POINT('Ctrl Pts',(16.6668554550744,-18.4952698494906,-8.73853791860778));
#84685=CARTESIAN_POINT('Ctrl Pts',(16.683415117402,-18.4203214021236,-8.74315074950144));
#84686=CARTESIAN_POINT('Ctrl Pts',(16.7040338351227,-18.3463705997984,-8.74776358039509));
#84687=CARTESIAN_POINT('Ctrl Pts',(16.7285569647209,-18.2738501402711,-8.75237641128874));
#84688=CARTESIAN_POINT('Ctrl Pts',(16.7531478646367,-18.2011292685346,-8.75700198986265));
#84689=CARTESIAN_POINT('Ctrl Pts',(16.7816645931624,-18.1298470190276,-8.76162756843655));
#84690=CARTESIAN_POINT('Ctrl Pts',(16.8139044122095,-18.060416053449,-8.76625314701046));
#84691=CARTESIAN_POINT('Ctrl Pts',(16.831243102243,-18.0230758317455,-8.76874079971725));
#84692=CARTESIAN_POINT('Ctrl Pts',(16.8496578472076,-17.9862706239721,-8.77122845242405));
#84693=CARTESIAN_POINT('Ctrl Pts',(16.8691118619909,-17.9500612629941,-8.77371610513084));
#84694=CARTESIAN_POINT('Ctrl Pts',(16.9034286623952,-17.8861881022462,-8.77810431406174));
#84695=CARTESIAN_POINT('Ctrl Pts',(16.9410977666969,-17.8239553476821,-8.78249252299263));
#84696=CARTESIAN_POINT('Ctrl Pts',(16.9819381659417,-17.7637372640547,-8.78688073192353));
#84697=CARTESIAN_POINT('Ctrl Pts',(17.0227179512625,-17.7036085540478,-8.79126242802479));
#84698=CARTESIAN_POINT('Ctrl Pts',(17.0666594195114,-17.6454889751329,-8.79564412412606));
#84699=CARTESIAN_POINT('Ctrl Pts',(17.1135357879719,-17.5897280970614,-8.80002582022733));
#84700=CARTESIAN_POINT('Ctrl Pts',(17.1603570729688,-17.5340327424593,-8.80440236748697));
#84701=CARTESIAN_POINT('Ctrl Pts',(17.2101060983649,-17.4806909501826,-8.80877891474661));
#84702=CARTESIAN_POINT('Ctrl Pts',(17.2625139124397,-17.4300217826406,-8.81315546200624));
#84703=CARTESIAN_POINT('Ctrl Pts',(17.3148884902405,-17.3793847487483,-8.81752923372322));
#84704=CARTESIAN_POINT('Ctrl Pts',(17.3699181652065,-17.331417311077,-8.82190300544019));
#84705=CARTESIAN_POINT('Ctrl Pts',(17.4272959551551,-17.2864029481336,-8.82627677715716));
#84706=CARTESIAN_POINT('Ctrl Pts',(17.4846562848495,-17.2414022832121,-8.83064921792072));
#84707=CARTESIAN_POINT('Ctrl Pts',(17.5443629316526,-17.1993532065252,-8.83502165868427));
#84708=CARTESIAN_POINT('Ctrl Pts',(17.6060758346833,-17.1604989318187,-8.83939409944782));
#84709=CARTESIAN_POINT('Ctrl Pts',(17.6677903157198,-17.1216436636041,-8.84376665201517));
#84710=CARTESIAN_POINT('Ctrl Pts',(17.7315107455603,-17.085983614876,-8.84813920458252));
#84711=CARTESIAN_POINT('Ctrl Pts',(17.7968695201138,-17.0537177597448,-8.85251175714986));
#84712=CARTESIAN_POINT('Ctrl Pts',(17.8622961264687,-17.0214184178922,-8.85688884771719));
#84713=CARTESIAN_POINT('Ctrl Pts',(17.9293640389057,-16.9925205167796,-8.86126593828452));
#84714=CARTESIAN_POINT('Ctrl Pts',(17.997683325039,-16.9671758883532,-8.86564302885184));
#84715=CARTESIAN_POINT('Ctrl Pts',(18.0660399228703,-16.9418174182846,-8.87002250991079));
#84716=CARTESIAN_POINT('Ctrl Pts',(18.135648794436,-16.9200162288388,-8.87440199096972));
#84717=CARTESIAN_POINT('Ctrl Pts',(18.2061050046724,-16.9018741809567,-8.87878147202867));
#84718=CARTESIAN_POINT('Ctrl Pts',(18.2766860980686,-16.8836999764164,-8.88316871568839));
#84719=CARTESIAN_POINT('Ctrl Pts',(18.348117056223,-16.869197961386,-8.88755595934811));
#84720=CARTESIAN_POINT('Ctrl Pts',(18.4199835016911,-16.8584187049962,-8.89194320300783));
#84721=CARTESIAN_POINT('Ctrl Pts',(18.4688457595752,-16.8510898493378,-8.89492610594264));
#84722=CARTESIAN_POINT('Ctrl Pts',(18.5179091821632,-16.8454808253817,-8.89790900887746));
#84723=CARTESIAN_POINT('Ctrl Pts',(18.567043338876,-16.8415937658104,-8.90089191181228));
#84724=CARTESIAN_POINT('Ctrl Pts',(18.6393255921073,-16.8358754337365,-8.90528012074317));
#84725=CARTESIAN_POINT('Ctrl Pts',(18.7120430618562,-16.8338637794812,-8.90966832967407));
#84726=CARTESIAN_POINT('Ctrl Pts',(18.7847830739803,-16.8356091855716,-8.91405653860496));
#84727=CARTESIAN_POINT('Ctrl Pts',(18.8574151278658,-16.8373520011898,-8.91843823470623));
#84728=CARTESIAN_POINT('Ctrl Pts',(18.9300691794578,-16.8428407963575,-8.9228199308075));
#84729=CARTESIAN_POINT('Ctrl Pts',(19.0023285427326,-16.8520740981751,-8.92720162690877));
#84730=CARTESIAN_POINT('Ctrl Pts',(19.074502995505,-16.8612965501284,-8.9315781741684));
#84731=CARTESIAN_POINT('Ctrl Pts',(19.1462832051701,-16.8742547070802,-8.93595472142804));
#84732=CARTESIAN_POINT('Ctrl Pts',(19.2172553122691,-16.8908951256271,-8.94033126868768));
#84733=CARTESIAN_POINT('Ctrl Pts',(19.2881824098894,-16.9075249910624,-8.94470504040465));
#84734=CARTESIAN_POINT('Ctrl Pts',(19.358301953298,-16.9278323748368,-8.94907881212162));
#84735=CARTESIAN_POINT('Ctrl Pts',(19.4272094182993,-16.9517125950551,-8.95345258383859));
#84736=CARTESIAN_POINT('Ctrl Pts',(19.4960959145276,-16.9755855484422,-8.95782502460214));
#84737=CARTESIAN_POINT('Ctrl Pts',(19.5637706090989,-17.0030290219352,-8.96219746536569));
#84738=CARTESIAN_POINT('Ctrl Pts',(19.6298449292375,-17.0338887251363,-8.96656990612924));
#84739=CARTESIAN_POINT('Ctrl Pts',(19.6959209389038,-17.0647492174234,-8.97094245869659));
#84740=CARTESIAN_POINT('Ctrl Pts',(19.7603960566782,-17.0990259069124,-8.97531501126393));
#84741=CARTESIAN_POINT('Ctrl Pts',(19.8229039996998,-17.1365173976494,-8.97968756383127));
#84742=CARTESIAN_POINT('Ctrl Pts',(19.8854768158224,-17.1740477984696,-8.9840646543986));
#84743=CARTESIAN_POINT('Ctrl Pts',(19.9460779664246,-17.2147994133216,-8.98844174496592));
#84744=CARTESIAN_POINT('Ctrl Pts',(20.004368721863,-17.25852655453,-8.99281883553325));
#84745=CARTESIAN_POINT('Ctrl Pts',(20.0626913120465,-17.3022775767531,-8.99719831659219));
#84746=CARTESIAN_POINT('Ctrl Pts',(20.1187006241991,-17.3490070515424,-9.00157779765113));
#84747=CARTESIAN_POINT('Ctrl Pts',(20.17209182572,-17.3984296279868,-9.00595727871007));
#84748=CARTESIAN_POINT('Ctrl Pts',(20.2255776627872,-17.4479398056161,-9.01034452236979));
#84749=CARTESIAN_POINT('Ctrl Pts',(20.2764357852878,-17.5001522715463,-9.01473176602951));
#84750=CARTESIAN_POINT('Ctrl Pts',(20.3243993779342,-17.5547459720343,-9.01911900968923));
#84751=CARTESIAN_POINT('Ctrl Pts',(20.3570099991731,-17.5918644277298,-9.02210191262405));
#84752=CARTESIAN_POINT('Ctrl Pts',(20.3882834007585,-17.6300829433876,-9.02508481555887));
#84753=CARTESIAN_POINT('Ctrl Pts',(20.4181471898432,-17.6692930019122,-9.0280677184937));
#84754=CARTESIAN_POINT('Ctrl Pts',(20.4620804149045,-17.7269757132704,-9.03245592742459));
#84755=CARTESIAN_POINT('Ctrl Pts',(20.5031324849612,-17.7870307272458,-9.03684413635549));
#84756=CARTESIAN_POINT('Ctrl Pts',(20.541037663595,-17.8491383212981,-9.04123234528639));
#84757=CARTESIAN_POINT('Ctrl Pts',(20.578886584659,-17.9111537373832,-9.04561404138766));
#84758=CARTESIAN_POINT('Ctrl Pts',(20.6135976366774,-17.9752152777401,-9.04999573748892));
#84759=CARTESIAN_POINT('Ctrl Pts',(20.6449465138838,-18.0409717781126,-9.05437743359019));
#84760=CARTESIAN_POINT('Ctrl Pts',(20.6762585536648,-18.1066510093641,-9.05875398084983));
#84761=CARTESIAN_POINT('Ctrl Pts',(20.7042160604134,-18.1740208108152,-9.06313052810947));
#84762=CARTESIAN_POINT('Ctrl Pts',(20.728639957299,-18.242704264255,-9.06750707536911));
#84763=CARTESIAN_POINT('Ctrl Pts',(20.7530483649043,-18.3113441596469,-9.07188084708609));
#84764=CARTESIAN_POINT('Ctrl Pts',(20.7739274477879,-18.3812956006723,-9.07625461880306));
#84765=CARTESIAN_POINT('Ctrl Pts',(20.7911462655829,-18.4521617841757,-9.08062839052004));
#84766=CARTESIAN_POINT('Ctrl Pts',(20.8083598436337,-18.5230064028614,-9.08500083128359));
#84767=CARTESIAN_POINT('Ctrl Pts',(20.8219152540694,-18.5947647429384,-9.08937327204714));
#84768=CARTESIAN_POINT('Ctrl Pts',(20.8317319036236,-18.6670265617294,-9.0937457128107));
#84769=CARTESIAN_POINT('Ctrl Pts',(20.8415488041906,-18.739290228263,-9.09811826537804));
#84770=CARTESIAN_POINT('Ctrl Pts',(20.847626691118,-18.8120569208142,-9.10249081794539));
#84771=CARTESIAN_POINT('Ctrl Pts',(20.8499366445659,-18.8849096416525,-9.10686337051273));
#84772=CARTESIAN_POINT('Ctrl Pts',(20.8522489953706,-18.9578379717924,-9.11124046108006));
#84773=CARTESIAN_POINT('Ctrl Pts',(20.8507855897922,-19.0308520253128,-9.11561755164739));
#84774=CARTESIAN_POINT('Ctrl Pts',(20.8455696643532,-19.1035339981098,-9.11999464221472));
#84775=CARTESIAN_POINT('Ctrl Pts',(20.8403508903038,-19.1762556652297,-9.12437412327366));
#84776=CARTESIAN_POINT('Ctrl Pts',(20.8313755754733,-19.2486444114932,-9.1287536043326));
#84777=CARTESIAN_POINT('Ctrl Pts',(20.8187186547149,-19.3202894658875,-9.13313308539154));
#84778=CARTESIAN_POINT('Ctrl Pts',(20.8060392996494,-19.3920615106598,-9.13752032905126));
#84779=CARTESIAN_POINT('Ctrl Pts',(20.789665415713,-19.4630867607306,-9.14190757271098));
#84780=CARTESIAN_POINT('Ctrl Pts',(20.769722536241,-19.532967086366,-9.14629481637071));
#84781=CARTESIAN_POINT('Ctrl Pts',(20.7561632998913,-19.5804789741458,-9.14927771930552));
#84782=CARTESIAN_POINT('Ctrl Pts',(20.7409552755656,-19.6274619134099,-9.15226062224033));
#84783=CARTESIAN_POINT('Ctrl Pts',(20.7241505240927,-19.6737962949846,-9.15524352517514));
#84784=CARTESIAN_POINT('Ctrl Pts',(20.6994287137937,-19.7419597422966,-9.15963173410604));
#84785=CARTESIAN_POINT('Ctrl Pts',(20.6711526578599,-19.8089846766148,-9.16401994303694));
#84786=CARTESIAN_POINT('Ctrl Pts',(20.6394473542677,-19.8744745959181,-9.16840815196783));
#84787=CARTESIAN_POINT('Ctrl Pts',(20.6077891066028,-19.9398673173227,-9.1727898480691));
#84788=CARTESIAN_POINT('Ctrl Pts',(20.5727119232316,-20.0037291156991,-9.17717154417037));
#84789=CARTESIAN_POINT('Ctrl Pts',(20.5343896652635,-20.0656813068433,-9.18155324027163));
#84790=CARTESIAN_POINT('Ctrl Pts',(20.4961124389984,-20.1275606992326,-9.18592978753127));
#84791=CARTESIAN_POINT('Ctrl Pts',(20.4545979656272,-20.187534533793,-9.19030633479091));
#84792=CARTESIAN_POINT('Ctrl Pts',(20.4100662428249,-20.2452482165706,-9.19468288205055));
#84793=CARTESIAN_POINT('Ctrl Pts',(20.3655627613939,-20.3029252981693,-9.19905665376752));
#84794=CARTESIAN_POINT('Ctrl Pts',(20.3180461211088,-20.3583446909811,-9.20343042548449));
#84795=CARTESIAN_POINT('Ctrl Pts',(20.2677790950909,-20.4111815128565,-9.20780419720147));
#84796=CARTESIAN_POINT('Ctrl Pts',(20.2175273654978,-20.4640022563096,-9.21217663796502));
#84797=CARTESIAN_POINT('Ctrl Pts',(20.1645272440667,-20.5142416397749,-9.21654907872857));
#84798=CARTESIAN_POINT('Ctrl Pts',(20.1090800563605,-20.5616098404892,-9.22092151949212));
#84799=CARTESIAN_POINT('Ctrl Pts',(20.0536314508636,-20.6089792524137,-9.22529407205947));
#84800=CARTESIAN_POINT('Ctrl Pts',(19.9957360229243,-20.6534770240217,-9.22966662462681));
#84801=CARTESIAN_POINT('Ctrl Pts',(19.9357287478819,-20.6948531253419,-9.23403917719415));
#84802=CARTESIAN_POINT('Ctrl Pts',(19.8756591950261,-20.7362721683408,-9.23841626776148));
#84803=CARTESIAN_POINT('Ctrl Pts',(19.8134738170561,-20.7745627981878,-9.24279335832881));
#84804=CARTESIAN_POINT('Ctrl Pts',(19.7495364985931,-20.8095184036841,-9.24717044889614));
#84805=CARTESIAN_POINT('Ctrl Pts',(19.6855642615875,-20.844493099734,-9.25154992995508));
#84806=CARTESIAN_POINT('Ctrl Pts',(19.61983861406,-20.8761289357272,-9.25592941101402));
#84807=CARTESIAN_POINT('Ctrl Pts',(19.552745510241,-20.9042665774582,-9.26030889207296));
#84808=CARTESIAN_POINT('Ctrl Pts',(19.4855334843459,-20.9324540929702,-9.26469613573268));
#84809=CARTESIAN_POINT('Ctrl Pts',(19.4169496162063,-20.957130868566,-9.2690833793924));
#84810=CARTESIAN_POINT('Ctrl Pts',(19.3473966187367,-20.9781869578404,-9.27347062305212));
#84811=CARTESIAN_POINT('Ctrl Pts',(19.3001072825683,-20.992503069587,-9.27645352598693));
#84812=CARTESIAN_POINT('Ctrl Pts',(19.2523702507339,-21.0051465017728,-9.27943642892175));
#84813=CARTESIAN_POINT('Ctrl Pts',(19.2043142751594,-21.0160962871391,-9.28241933185657));
#84814=CARTESIAN_POINT('Ctrl Pts',(19.1336181560407,-21.0322047381968,-9.28680754078747));
#84815=CARTESIAN_POINT('Ctrl Pts',(19.0619555004258,-21.0447083756574,-9.29119574971836));
#84816=CARTESIAN_POINT('Ctrl Pts',(18.9897273628003,-21.0534976840138,-9.29558395864926));
#84817=CARTESIAN_POINT('Ctrl Pts',(18.9176064237068,-21.0622739475792,-9.29996565475053));
#84818=CARTESIAN_POINT('Ctrl Pts',(18.8449221435535,-21.0673467676749,-9.30434735085179));
#84819=CARTESIAN_POINT('Ctrl Pts',(18.772087043549,-21.0686573594027,-9.30872904695306));
#84820=CARTESIAN_POINT('Ctrl Pts',(18.6993375305834,-21.0699664110809,-9.3131055942127));
#84821=CARTESIAN_POINT('Ctrl Pts',(18.6264380297317,-21.0675220079374,-9.31748214147234));
#84822=CARTESIAN_POINT('Ctrl Pts',(18.5538057789621,-21.0613171982195,-9.32185868873198));
#84823=CARTESIAN_POINT('Ctrl Pts',(18.4812195905103,-21.0551163235017,-9.32623246044895));
#84824=CARTESIAN_POINT('Ctrl Pts',(18.4089007953027,-21.0451598149104,-9.33060623216593));
#84825=CARTESIAN_POINT('Ctrl Pts',(18.3372648019199,-21.0314927705102,-9.3349800038829));
#84826=CARTESIAN_POINT('Ctrl Pts',(18.2656506076104,-21.0178298850376,-9.33935244464645));
#84827=CARTESIAN_POINT('Ctrl Pts',(18.194719276167,-21.0004587957696,-9.34372488541));
#84828=CARTESIAN_POINT('Ctrl Pts',(18.1248776044803,-20.979475994254,-9.34809732617356));
#84829=CARTESIAN_POINT('Ctrl Pts',(18.0550341469343,-20.9584926562059,-9.3524698787409));
#84830=CARTESIAN_POINT('Ctrl Pts',(17.9862808658671,-20.9338975632636,-9.35684243130824));
#84831=CARTESIAN_POINT('Ctrl Pts',(17.9190093127144,-20.9058370401949,-9.36121498387559));
#84832=CARTESIAN_POINT('Ctrl Pts',(17.8516679426063,-20.877747394857,-9.36559207444291));
#84833=CARTESIAN_POINT('Ctrl Pts',(17.7858118168723,-20.8461853247306,-9.36996916501024));
#84834=CARTESIAN_POINT('Ctrl Pts',(17.7218116266775,-20.8113449644729,-9.37434625557757));
#84835=CARTESIAN_POINT('Ctrl Pts',(17.6577764836036,-20.7764855766014,-9.37872573663651));
#84836=CARTESIAN_POINT('Ctrl Pts',(17.5955997055917,-20.738344586342,-9.38310521769546));
#84837=CARTESIAN_POINT('Ctrl Pts',(17.5356241771984,-20.6971602755405,-9.3874846987544));
#84838=CARTESIAN_POINT('Ctrl Pts',(17.4755423425837,-20.6559029658246,-9.39187194241412));
#84839=CARTESIAN_POINT('Ctrl Pts',(17.417669932464,-20.6115918569496,-9.39625918607384));
#84840=CARTESIAN_POINT('Ctrl Pts',(17.3623173752293,-20.564506054842,-9.40064642973356));
#84841=CARTESIAN_POINT('Ctrl Pts',(17.3246829700694,-20.532492246586,-9.40362933266838));
#84842=CARTESIAN_POINT('Ctrl Pts',(17.2882126945401,-20.4991966074029,-9.40661223560319));
#84843=CARTESIAN_POINT('Ctrl Pts',(17.2529938697634,-20.4647160481073,-9.40959513853801));
#84844=CARTESIAN_POINT('Ctrl Pts',(17.201926340437,-20.4147190086213,-9.41392036756161));
#84845=CARTESIAN_POINT('Ctrl Pts',(17.153279990606,-20.3620217118529,-9.41824559658522));
#84846=CARTESIAN_POINT('Ctrl Pts',(17.1073599831676,-20.3068916029112,-9.42257082560882));
#84847=CARTESIAN_POINT('Ctrl Pts',(17.0615168757444,-20.2518538176963,-9.4268888113806));
#84848=CARTESIAN_POINT('Ctrl Pts',(17.0183913618816,-20.194391687294,-9.43120679715237));
#84849=CARTESIAN_POINT('Ctrl Pts',(16.9782524640737,-20.1348100397311,-9.43552478292415));
#84850=CARTESIAN_POINT('Ctrl Pts',(16.9381523085283,-20.075285900669,-9.43983860095472));
#84851=CARTESIAN_POINT('Ctrl Pts',(16.9010333312299,-20.0136467098988,-9.44415241898528));
#84852=CARTESIAN_POINT('Ctrl Pts',(16.8671239501054,-19.9502298404326,-9.44846623701585));
#84853=CARTESIAN_POINT('Ctrl Pts',(16.8332351489702,-19.886851459386,-9.45277743694118));
#84854=CARTESIAN_POINT('Ctrl Pts',(16.8025523148356,-19.8216979770288,-9.4570886368665));
#84855=CARTESIAN_POINT('Ctrl Pts',(16.7752592184707,-19.755133582148,-9.46139983679183));
#84856=CARTESIAN_POINT('Ctrl Pts',(16.7648137941534,-19.729658519163,-9.46304978929024));
#84857=CARTESIAN_POINT('Ctrl Pts',(16.7548643808522,-19.7039770531934,-9.46469974178865));
#84858=CARTESIAN_POINT('Ctrl Pts',(16.7454194499637,-19.6781104571739,-9.46634969428706));
#84859=CARTESIAN_POINT('',(16.6170008950802,-18.9500532671891,-8.48905627902251));
#84860=CARTESIAN_POINT('Ctrl Pts',(16.7454193049359,-19.6781100599899,-9.24346979696294));
#84861=CARTESIAN_POINT('Ctrl Pts',(16.7776919679286,-19.7664944498252,-9.23734829963788));
#84862=CARTESIAN_POINT('Ctrl Pts',(16.8158509947677,-19.8527102299079,-9.23135282091049));
#84863=CARTESIAN_POINT('Ctrl Pts',(16.870699146144,-19.9571673936568,-9.22408567207777));
#84864=CARTESIAN_POINT('Ctrl Pts',(16.8820779974327,-19.9779807646683,-9.22263707125759));
#84865=CARTESIAN_POINT('Ctrl Pts',(16.8985836849794,-20.0070020846846,-9.22061560073741));
#84866=CARTESIAN_POINT('Ctrl Pts',(16.9034203307547,-20.0153722431622,-9.22003238534716));
#84867=CARTESIAN_POINT('Ctrl Pts',(16.9113459968973,-20.0288738325939,-9.21909122021068));
#84868=CARTESIAN_POINT('Ctrl Pts',(16.9143997169755,-20.0340257286749,-9.21873199734405));
#84869=CARTESIAN_POINT('Ctrl Pts',(16.9208165154469,-20.0447474470033,-9.21798418043392));
#84870=CARTESIAN_POINT('Ctrl Pts',(16.9241834957213,-20.0503148701018,-9.21759573377162));
#84871=CARTESIAN_POINT('Ctrl Pts',(16.9322157277914,-20.0634592247858,-9.21667827532294));
#84872=CARTESIAN_POINT('Ctrl Pts',(16.9369032114755,-20.0710224789062,-9.21615008615486));
#84873=CARTESIAN_POINT('Ctrl Pts',(16.9526728496646,-20.0961121277849,-9.21439677543285));
#84874=CARTESIAN_POINT('Ctrl Pts',(16.9639650239576,-20.1135055772994,-9.21317942997755));
#84875=CARTESIAN_POINT('Ctrl Pts',(17.0256090451949,-20.2054691714003,-9.20672827219186));
#84876=CARTESIAN_POINT('Ctrl Pts',(17.0804235748791,-20.2769423779121,-9.20166741840291));
#84877=CARTESIAN_POINT('Ctrl Pts',(17.2287762363623,-20.4467756329287,-9.18922995126064));
#84878=CARTESIAN_POINT('Ctrl Pts',(17.3275154071975,-20.5400338848918,-9.18201734532298));
#84879=CARTESIAN_POINT('Ctrl Pts',(17.4939965849843,-20.6694875077123,-9.17034163101494));
#84880=CARTESIAN_POINT('Ctrl Pts',(17.5559297040637,-20.7125452644636,-9.16608158963595));
#84881=CARTESIAN_POINT('Ctrl Pts',(17.628088335483,-20.7571976182767,-9.16105236809672));
#84882=CARTESIAN_POINT('Ctrl Pts',(17.6361911110664,-20.7621366485825,-9.16048672412422));
#84883=CARTESIAN_POINT('Ctrl Pts',(17.6482528193402,-20.7693780648497,-9.15964295207999));
#84884=CARTESIAN_POINT('Ctrl Pts',(17.6521865875829,-20.7717224268327,-9.15936749146939));
#84885=CARTESIAN_POINT('Ctrl Pts',(17.6592019909693,-20.7758725276173,-9.15887569444401));
#84886=CARTESIAN_POINT('Ctrl Pts',(17.6622806197075,-20.7776832493309,-9.15865968652276));
#84887=CARTESIAN_POINT('Ctrl Pts',(17.6689127423215,-20.7815614323407,-9.15819393177831));
#84888=CARTESIAN_POINT('Ctrl Pts',(17.6724676284311,-20.7836263059437,-9.15794402899267));
#84889=CARTESIAN_POINT('Ctrl Pts',(17.6823047444223,-20.7893019877147,-9.15725184545361));
#84890=CARTESIAN_POINT('Ctrl Pts',(17.688599463882,-20.7928908767911,-9.15680819102671));
#84891=CARTESIAN_POINT('Ctrl Pts',(17.7233171356835,-20.8124494202391,-9.15435780236056));
#84892=CARTESIAN_POINT('Ctrl Pts',(17.7520859964798,-20.8277922370323,-9.15231457852842));
#84893=CARTESIAN_POINT('Ctrl Pts',(17.9264392723837,-20.9156672650139,-9.139907154325));
#84894=CARTESIAN_POINT('Ctrl Pts',(18.0796307715685,-20.9718872018195,-9.12895410545955));
#84895=CARTESIAN_POINT('Ctrl Pts',(18.3512845860962,-21.0373916249034,-9.11070140547799));
#84896=CARTESIAN_POINT('Ctrl Pts',(18.4669069766484,-21.0553303203647,-9.1032618877738));
#84897=CARTESIAN_POINT('Ctrl Pts',(18.5976892024241,-21.0646553302264,-9.09525606163682));
#84898=CARTESIAN_POINT('Ctrl Pts',(18.6119522891808,-21.0655272768218,-9.09438810180259));
#84899=CARTESIAN_POINT('Ctrl Pts',(18.6346668639344,-21.0666851788318,-9.09301381397604));
#84900=CARTESIAN_POINT('Ctrl Pts',(18.6431129331723,-21.067065015978,-9.09250455805295));
#84901=CARTESIAN_POINT('Ctrl Pts',(18.6580129559602,-21.0676456835164,-9.09160918539496));
#84902=CARTESIAN_POINT('Ctrl Pts',(18.6644659349539,-21.0678676008376,-9.09122241255801));
#84903=CARTESIAN_POINT('Ctrl Pts',(18.6778149090636,-21.0682655360733,-9.09042434286681));
#84904=CARTESIAN_POINT('Ctrl Pts',(18.6847109590881,-21.0684373781884,-9.09001318140611));
#84905=CARTESIAN_POINT('Ctrl Pts',(18.7024144118008,-21.0687919549537,-9.08896046175823));
#84906=CARTESIAN_POINT('Ctrl Pts',(18.7132226813714,-21.0689256339154,-9.08832044492973));
#84907=CARTESIAN_POINT('Ctrl Pts',(18.7583376119597,-21.0691380695254,-9.08565970126129));
#84908=CARTESIAN_POINT('Ctrl Pts',(18.7926437411782,-21.0684656937997,-9.0836625049292));
#84909=CARTESIAN_POINT('Ctrl Pts',(18.881974433319,-21.0645409869583,-9.07851821178175));
#84910=CARTESIAN_POINT('Ctrl Pts',(18.9369160470631,-21.0599733342275,-9.07541050829213));
#84911=CARTESIAN_POINT('Ctrl Pts',(19.1001558930883,-21.0399597647981,-9.06626584573491));
#84912=CARTESIAN_POINT('Ctrl Pts',(19.2075006717982,-21.0182633217052,-9.0603776152195));
#84913=CARTESIAN_POINT('Ctrl Pts',(19.3568854813903,-20.9758117003682,-9.05192244406373));
#84914=CARTESIAN_POINT('Ctrl Pts',(19.4006606512077,-20.9618167718137,-9.04941010653216));
#84915=CARTESIAN_POINT('Ctrl Pts',(19.4649346690079,-20.9389373236352,-9.0456264925304));
#84916=CARTESIAN_POINT('Ctrl Pts',(19.4858051398379,-20.9311347608811,-9.04438268387586));
#84917=CARTESIAN_POINT('Ctrl Pts',(19.5544069538365,-20.9042458326511,-9.04023204677506));
#84918=CARTESIAN_POINT('Ctrl Pts',(19.6015626744835,-20.8837519108841,-9.0372783279366));
#84919=CARTESIAN_POINT('Ctrl Pts',(19.6550271847821,-20.858163680944,-9.03376033623064));
#84920=CARTESIAN_POINT('Ctrl Pts',(19.6621135638716,-20.8547233802766,-9.03329054236549));
#84921=CARTESIAN_POINT('Ctrl Pts',(19.6733812317493,-20.8491752229195,-9.03253768384218));
#84922=CARTESIAN_POINT('Ctrl Pts',(19.677575090663,-20.8470928664156,-9.03225616440731));
#84923=CARTESIAN_POINT('Ctrl Pts',(19.6849748640897,-20.8433880400916,-9.03175707545887));
#84924=CARTESIAN_POINT('Ctrl Pts',(19.6881835993648,-20.8417713006821,-9.0315398658903));
#84925=CARTESIAN_POINT('Ctrl Pts',(19.6949586570297,-20.8383359946607,-9.0310795427533));
#84926=CARTESIAN_POINT('Ctrl Pts',(19.6985238859734,-20.8365155075098,-9.03083631431778));
#84927=CARTESIAN_POINT('Ctrl Pts',(19.7080942340707,-20.8315943974037,-9.0301807723508));
#84928=CARTESIAN_POINT('Ctrl Pts',(19.714089645224,-20.8284751424081,-9.02976731099744));
#84929=CARTESIAN_POINT('Ctrl Pts',(19.7432925091862,-20.8131035273658,-9.02774010670412));
#84930=CARTESIAN_POINT('Ctrl Pts',(19.7662845820032,-20.8004496487409,-9.02610292272586));
#84931=CARTESIAN_POINT('Ctrl Pts',(19.8314666132126,-20.7629808081381,-9.02135531277092));
#84932=CARTESIAN_POINT('Ctrl Pts',(19.8730376703919,-20.7371266082566,-9.01819732379401));
#84933=CARTESIAN_POINT('Ctrl Pts',(19.993928502925,-20.6559985117303,-9.00869694294965));
#84934=CARTESIAN_POINT('Ctrl Pts',(20.0704008099772,-20.5967077052518,-9.00226771860933));
#84935=CARTESIAN_POINT('Ctrl Pts',(20.2478287560177,-20.4385725247757,-8.98663170183146));
#84936=CARTESIAN_POINT('Ctrl Pts',(20.3434811410304,-20.3344468098612,-8.97756399134499));
#84937=CARTESIAN_POINT('Ctrl Pts',(20.4366435908121,-20.210132659946,-8.96807848728317));
#84938=CARTESIAN_POINT('Ctrl Pts',(20.4450930131601,-20.1986169032086,-8.96721093793812));
#84939=CARTESIAN_POINT('Ctrl Pts',(20.4583564388408,-20.1801511782516,-8.96583717516303));
#84940=CARTESIAN_POINT('Ctrl Pts',(20.4632463588114,-20.1732565162926,-8.96532803728183));
#84941=CARTESIAN_POINT('Ctrl Pts',(20.4717983602435,-20.1610440620952,-8.96443280191692));
#84942=CARTESIAN_POINT('Ctrl Pts',(20.4754776284878,-20.1557384914763,-8.96404604896419));
#84943=CARTESIAN_POINT('Ctrl Pts',(20.4830379944307,-20.1447290926685,-8.96324795301442));
#84944=CARTESIAN_POINT('Ctrl Pts',(20.4869156019338,-20.1390229520482,-8.96283674574297));
#84945=CARTESIAN_POINT('Ctrl Pts',(20.4967986457271,-20.1243253993542,-8.96178376947603));
#84946=CARTESIAN_POINT('Ctrl Pts',(20.5027632638387,-20.1153066794308,-8.96114354331472));
#84947=CARTESIAN_POINT('Ctrl Pts',(20.52738030171,-20.0774577550668,-8.95848076421811));
#84948=CARTESIAN_POINT('Ctrl Pts',(20.545399614189,-20.0482206437836,-8.95648178776577));
#84949=CARTESIAN_POINT('Ctrl Pts',(20.5904987951057,-19.9708943430114,-8.95133187211742));
#84950=CARTESIAN_POINT('Ctrl Pts',(20.6164243625228,-19.9221611337104,-8.94822043926862));
#84951=CARTESIAN_POINT('Ctrl Pts',(20.6879870509115,-19.7739447883822,-8.93906927114948));
#84952=CARTESIAN_POINT('Ctrl Pts',(20.7278487032641,-19.6718797507182,-8.93317824260384));
#84953=CARTESIAN_POINT('Ctrl Pts',(20.7744408176174,-19.5184657484256,-8.92444873437601));
#84954=CARTESIAN_POINT('Ctrl Pts',(20.7874754897926,-19.4692235853106,-8.92166296549719));
#84955=CARTESIAN_POINT('Ctrl Pts',(20.8021906400655,-19.40424238805,-8.91795609658116));
#84956=CARTESIAN_POINT('Ctrl Pts',(20.8054889807911,-19.3888856673185,-8.91707782644251));
#84957=CARTESIAN_POINT('Ctrl Pts',(20.8191178653758,-19.321803557602,-8.91322621815388));
#84958=CARTESIAN_POINT('Ctrl Pts',(20.8276832231,-19.2697432242618,-8.91019826366661));
#84959=CARTESIAN_POINT('Ctrl Pts',(20.8353850229457,-19.2087986388804,-8.9065526623584));
#84960=CARTESIAN_POINT('Ctrl Pts',(20.836421686752,-19.2001684927691,-8.90603407633398));
#84961=CARTESIAN_POINT('Ctrl Pts',(20.8379117366104,-19.1870839210295,-8.90524394221665));
#84962=CARTESIAN_POINT('Ctrl Pts',(20.8384042008505,-19.1826339176486,-8.90497454194854));
#84963=CARTESIAN_POINT('Ctrl Pts',(20.8392632772108,-19.1746392435701,-8.90448927664491));
#84964=CARTESIAN_POINT('Ctrl Pts',(20.839635058539,-19.1710951827401,-8.90427370566166));
#84965=CARTESIAN_POINT('Ctrl Pts',(20.8404239563872,-19.1633873841434,-8.90380387821813));
#84966=CARTESIAN_POINT('Ctrl Pts',(20.8408376712661,-19.1592233974523,-8.90354943881656));
#84967=CARTESIAN_POINT('Ctrl Pts',(20.8419662917948,-19.1475111267443,-8.90283206069093));
#84968=CARTESIAN_POINT('Ctrl Pts',(20.8426529866115,-19.1399602779432,-8.90236758282333));
#84969=CARTESIAN_POINT('Ctrl Pts',(20.8465378362426,-19.0945387942675,-8.89956227505961));
#84970=CARTESIAN_POINT('Ctrl Pts',(20.8487560451338,-19.0565938410345,-8.89717169067059));
#84971=CARTESIAN_POINT('Ctrl Pts',(20.8527120495246,-18.9309312712568,-8.88914350123471));
#84972=CARTESIAN_POINT('Ctrl Pts',(20.8500194730265,-18.8431685016411,-8.88336090965856));
#84973=CARTESIAN_POINT('Ctrl Pts',(20.825729171169,-18.5821608169637,-8.86604055244744));
#84974=CARTESIAN_POINT('Ctrl Pts',(20.7881616998726,-18.4111167304525,-8.85459338872171));
#84975=CARTESIAN_POINT('Ctrl Pts',(20.7223353808918,-18.2248525273578,-8.84243270523744));
#84976=CARTESIAN_POINT('Ctrl Pts',(20.714294527328,-18.2032312206241,-8.84102454648127));
#84977=CARTESIAN_POINT('Ctrl Pts',(20.7024238956251,-18.1728416523365,-8.83904951700229));
#84978=CARTESIAN_POINT('Ctrl Pts',(20.698885827654,-18.1639618964964,-8.83847292654427));
#84979=CARTESIAN_POINT('Ctrl Pts',(20.6930407959344,-18.1495763031934,-8.83753956930673));
#84980=CARTESIAN_POINT('Ctrl Pts',(20.6907705019473,-18.1440557982293,-8.83718157032278));
#84981=CARTESIAN_POINT('Ctrl Pts',(20.6859705802597,-18.1325230950597,-8.83643403188766));
#84982=CARTESIAN_POINT('Ctrl Pts',(20.6834364509379,-18.1265128292017,-8.83604464979026));
#84983=CARTESIAN_POINT('Ctrl Pts',(20.6773439849278,-18.1122476802427,-8.83512088673321));
#84984=CARTESIAN_POINT('Ctrl Pts',(20.6737607510275,-18.1040035171879,-8.83458735986114));
#84985=CARTESIAN_POINT('Ctrl Pts',(20.6615229506852,-18.0763307502198,-8.83279743296948));
#84986=CARTESIAN_POINT('Ctrl Pts',(20.6526279629415,-18.0570094141352,-8.83154926868361));
#84987=CARTESIAN_POINT('Ctrl Pts',(20.5767423400352,-17.8985066588994,-8.82131512662616));
#84988=CARTESIAN_POINT('Ctrl Pts',(20.4949941348804,-17.7669030984535,-8.81289767166638));
#84989=CARTESIAN_POINT('Ctrl Pts',(20.3152266158616,-17.5377449928549,-8.79708097714466));
#84990=CARTESIAN_POINT('Ctrl Pts',(20.2205923616352,-17.438584127056,-8.78969553452319));
#84991=CARTESIAN_POINT('Ctrl Pts',(20.105275088571,-17.3390720501843,-8.78076350845691));
#84992=CARTESIAN_POINT('Ctrl Pts',(20.0933630792143,-17.3290200473233,-8.77984139796247));
#84993=CARTESIAN_POINT('Ctrl Pts',(20.0768874921386,-17.3154256726584,-8.77856503898545));
#84994=CARTESIAN_POINT('Ctrl Pts',(20.0724184651143,-17.3117688102227,-8.77821872732565));
#84995=CARTESIAN_POINT('Ctrl Pts',(20.065288234416,-17.305982912755,-8.77766593871028));
#84996=CARTESIAN_POINT('Ctrl Pts',(20.0626367164115,-17.3038419098822,-8.77746031732908));
#84997=CARTESIAN_POINT('Ctrl Pts',(20.057145634574,-17.2994299257566,-8.77703434926696));
#84998=CARTESIAN_POINT('Ctrl Pts',(20.0543053941631,-17.29715986091,-8.7768139373675));
#84999=CARTESIAN_POINT('Ctrl Pts',(20.0475167861269,-17.2917626611136,-8.77628694959207));
#85000=CARTESIAN_POINT('Ctrl Pts',(20.0435630911632,-17.2886422880421,-8.77597989611487));
#85001=CARTESIAN_POINT('Ctrl Pts',(20.0301589952398,-17.2781407912089,-8.77493855608421));
#85002=CARTESIAN_POINT('Ctrl Pts',(20.0206572296242,-17.2708260203101,-8.77419980372735));
#85003=CARTESIAN_POINT('Ctrl Pts',(19.9093861176051,-17.1866616909484,-8.76554694658337));
#85004=CARTESIAN_POINT('Ctrl Pts',(19.8009453235383,-17.1190862529271,-8.75711389995272));
#85005=CARTESIAN_POINT('Ctrl Pts',(19.5397089949247,-16.9873707398854,-8.73778010492853));
#85006=CARTESIAN_POINT('Ctrl Pts',(19.3841063340161,-16.9305360372442,-8.72698434280298));
#85007=CARTESIAN_POINT('Ctrl Pts',(19.2004906969226,-16.8869012971584,-8.71536072261149));
#85008=CARTESIAN_POINT('Ctrl Pts',(19.1774343424353,-16.8818279594354,-8.71391911587544));
#85009=CARTESIAN_POINT('Ctrl Pts',(19.1448412695825,-16.8752256899708,-8.71190568322891));
#85010=CARTESIAN_POINT('Ctrl Pts',(19.1353722358856,-16.8733748734631,-8.71132362107856));
#85011=CARTESIAN_POINT('Ctrl Pts',(19.120008820235,-16.8704808395037,-8.71038381615215));
#85012=CARTESIAN_POINT('Ctrl Pts',(19.1141221656495,-16.8693977899901,-8.71002480740888));
#85013=CARTESIAN_POINT('Ctrl Pts',(19.1018244426444,-16.8671890861126,-8.70927704567564));
#85014=CARTESIAN_POINT('Ctrl Pts',(19.0954126087906,-16.8660680032807,-8.70888844178058));
#85015=CARTESIAN_POINT('Ctrl Pts',(19.0802085013706,-16.8634818359437,-8.70796991305197));
#85016=CARTESIAN_POINT('Ctrl Pts',(19.0714118998477,-16.8620426651347,-8.70744081617181));
#85017=CARTESIAN_POINT('Ctrl Pts',(19.0426186522532,-16.8575184651841,-8.70571639578555));
#85018=CARTESIAN_POINT('Ctrl Pts',(19.0225864536086,-16.8546644825232,-8.70452838408815));
#85019=CARTESIAN_POINT('Ctrl Pts',(18.974920071101,-16.848569349772,-8.70172733448518));
#85020=CARTESIAN_POINT('Ctrl Pts',(18.9472565402445,-16.8455848630125,-8.70012225584048));
#85021=CARTESIAN_POINT('Ctrl Pts',(18.7508329874053,-16.8283031137888,-8.68885155263308));
#85022=CARTESIAN_POINT('Ctrl Pts',(18.5809584419909,-16.8337571618947,-8.67982435317146));
#85023=CARTESIAN_POINT('Ctrl Pts',(18.310787758827,-16.8751305967414,-8.66488752605422));
#85024=CARTESIAN_POINT('Ctrl Pts',(18.2093449552684,-16.898411345124,-8.65912326062646));
#85025=CARTESIAN_POINT('Ctrl Pts',(18.1007796340158,-16.9318973238039,-8.65239231633011));
#85026=CARTESIAN_POINT('Ctrl Pts',(18.0915420562897,-16.9348161618779,-8.65181500406995));
#85027=CARTESIAN_POINT('Ctrl Pts',(18.0779311512388,-16.9392198349403,-8.65095713553893));
#85028=CARTESIAN_POINT('Ctrl Pts',(18.0735419767694,-16.9406557913186,-8.65067937776165));
#85029=CARTESIAN_POINT('Ctrl Pts',(18.0657629053151,-16.9432289901408,-8.65018505739779));
#85030=CARTESIAN_POINT('Ctrl Pts',(18.0623711540428,-16.9443604711422,-8.64996883632028));
#85031=CARTESIAN_POINT('Ctrl Pts',(18.0551094912353,-16.9468034079696,-8.64950440934813));
#85032=CARTESIAN_POINT('Ctrl Pts',(18.0512405635853,-16.9481174568066,-8.64925605686877));
#85033=CARTESIAN_POINT('Ctrl Pts',(18.0406289366111,-16.9517559059967,-8.64857242336353));
#85034=CARTESIAN_POINT('Ctrl Pts',(18.0338942138201,-16.9541031678388,-8.64813582291551));
#85035=CARTESIAN_POINT('Ctrl Pts',(17.9984775044218,-16.9666480640225,-8.64582590065809));
#85036=CARTESIAN_POINT('Ctrl Pts',(17.9700076578876,-16.9774288745619,-8.64392087630941));
#85037=CARTESIAN_POINT('Ctrl Pts',(17.7914210963493,-17.0494953350584,-8.63170745259291));
#85038=CARTESIAN_POINT('Ctrl Pts',(17.6485335844143,-17.1272422377809,-8.62079146652433));
#85039=CARTESIAN_POINT('Ctrl Pts',(17.4180930488449,-17.2893560683257,-8.60236920542641));
#85040=CARTESIAN_POINT('Ctrl Pts',(17.3262604599594,-17.3663538582294,-8.59474158434334));
#85041=CARTESIAN_POINT('Ctrl Pts',(17.2302711945353,-17.4617867664482,-8.58647638876815));
#85042=CARTESIAN_POINT('Ctrl Pts',(17.2192537691698,-17.4729869240252,-8.58552258211336));
#85043=CARTESIAN_POINT('Ctrl Pts',(17.2027731923366,-17.490118184151,-8.58408765426244));
#85044=CARTESIAN_POINT('Ctrl Pts',(17.1972177503297,-17.495959375594,-8.58360251642554));
#85045=CARTESIAN_POINT('Ctrl Pts',(17.1873222630543,-17.5064835730841,-8.58273572702831));
#85046=CARTESIAN_POINT('Ctrl Pts',(17.1829698067502,-17.5111547260519,-8.58235354278634));
#85047=CARTESIAN_POINT('Ctrl Pts',(17.1737790493218,-17.5211083560604,-8.58154448373944));
#85048=CARTESIAN_POINT('Ctrl Pts',(17.1689462847743,-17.5263958536727,-8.58111784772801));
#85049=CARTESIAN_POINT('Ctrl Pts',(17.1591629011719,-17.5372095009902,-8.58025163733869));
#85050=CARTESIAN_POINT('Ctrl Pts',(17.1542143063962,-17.54273735296,-8.57981215120182));
#85051=CARTESIAN_POINT('Ctrl Pts',(17.132425659083,-17.5673354613014,-8.57787095716848));
#85052=CARTESIAN_POINT('Ctrl Pts',(17.1159006593686,-17.5866828719498,-8.57638235546039));
#85053=CARTESIAN_POINT('Ctrl Pts',(17.0457286191984,-17.6719041411568,-8.56998123517883));
#85054=CARTESIAN_POINT('Ctrl Pts',(16.9957224890905,-17.7406787534278,-8.56521401094969));
#85055=CARTESIAN_POINT('Ctrl Pts',(16.9128101522339,-17.8704624229312,-8.55672636428035));
#85056=CARTESIAN_POINT('Ctrl Pts',(16.8785074359584,-17.9304307705728,-8.55298123350471));
#85057=CARTESIAN_POINT('Ctrl Pts',(16.7878577129973,-18.108589850488,-8.54212537034257));
#85058=CARTESIAN_POINT('Ctrl Pts',(16.7394673001256,-18.2304457765856,-8.53503483493165));
#85059=CARTESIAN_POINT('Ctrl Pts',(16.6982006722164,-18.3710882901915,-8.52644200352335));
#85060=CARTESIAN_POINT('Ctrl Pts',(16.6939331602486,-18.3862575020306,-8.52550990850784));
#85061=CARTESIAN_POINT('Ctrl Pts',(16.6883270785526,-18.4070734496436,-8.52422183350569));
#85062=CARTESIAN_POINT('Ctrl Pts',(16.6868416776032,-18.4126805695452,-8.52387397958134));
#85063=CARTESIAN_POINT('Ctrl Pts',(16.6845188928767,-18.4215965300107,-8.52331933758435));
#85064=CARTESIAN_POINT('Ctrl Pts',(16.6836664224205,-18.4249014611092,-8.52311341540417));
#85065=CARTESIAN_POINT('Ctrl Pts',(16.6819231281433,-18.4317282354038,-8.52268734811974));
#85066=CARTESIAN_POINT('Ctrl Pts',(16.6810333787528,-18.4352503040055,-8.52246714014281));
#85067=CARTESIAN_POINT('Ctrl Pts',(16.6789361654079,-18.4436430218554,-8.52194150042947));
#85068=CARTESIAN_POINT('Ctrl Pts',(16.6777369494926,-18.4485156929909,-8.52163559751192));
#85069=CARTESIAN_POINT('Ctrl Pts',(16.675232597529,-18.4588496058647,-8.5209853740746));
#85070=CARTESIAN_POINT('Ctrl Pts',(16.6739318448418,-18.4643118586532,-8.52064081548478));
#85071=CARTESIAN_POINT('Ctrl Pts',(16.6704195265389,-18.4793259488364,-8.51969147306472));
#85072=CARTESIAN_POINT('Ctrl Pts',(16.6682525934496,-18.4888879472955,-8.51908436631309));
#85073=CARTESIAN_POINT('Ctrl Pts',(16.6336164634003,-18.646807751159,-8.50902048411727));
#85074=CARTESIAN_POINT('Ctrl Pts',(16.6171414698365,-18.7982035803618,-8.49886432225171));
#85075=CARTESIAN_POINT('Ctrl Pts',(16.6170009071471,-18.950040188799,-8.48885784002949));
#85076=CARTESIAN_POINT('Ctrl Pts',(16.6170008950802,-18.9500532671891,-8.48905627902251));
#85077=CARTESIAN_POINT('Ctrl Pts',(16.6169347305481,-19.0220047205615,-8.48473008583426));
#85078=CARTESIAN_POINT('Ctrl Pts',(16.6205409900205,-19.09405109857,-8.48040389264601));
#85079=CARTESIAN_POINT('Ctrl Pts',(16.6278220014955,-19.1657831579326,-8.47607769945775));
#85080=CARTESIAN_POINT('Ctrl Pts',(16.6350980157525,-19.2374659850227,-8.47175447549029));
#85081=CARTESIAN_POINT('Ctrl Pts',(16.6460437282404,-19.3088344307521,-8.46743125152283));
#85082=CARTESIAN_POINT('Ctrl Pts',(16.6606094541866,-19.3794817476005,-8.46310802755537));
#85083=CARTESIAN_POINT('Ctrl Pts',(16.6751723924897,-19.4501155437014,-8.45878563098267));
#85084=CARTESIAN_POINT('Ctrl Pts',(16.6933538757661,-19.520027999392,-8.45446323440996));
#85085=CARTESIAN_POINT('Ctrl Pts',(16.7150529432357,-19.5888216249334,-8.45014083783726));
#85086=CARTESIAN_POINT('Ctrl Pts',(16.7245112166523,-19.6188076563883,-8.44825677490891));
#85087=CARTESIAN_POINT('Ctrl Pts',(16.7346371622268,-19.6485812753992,-8.44637271198055));
#85088=CARTESIAN_POINT('Ctrl Pts',(16.7454194499637,-19.6781104571739,-8.4444886490522));
#85089=CARTESIAN_POINT('Origin',(18.734,-18.952,0.));
#85090=CARTESIAN_POINT('',(16.7430902533864,-19.6789409674447,-7.64456001990001));
#85091=CARTESIAN_POINT('',(16.7454194590822,-19.6781104821466,-7.86510586795993));
#85092=CARTESIAN_POINT('',(16.7454194499637,-19.6781104571739,0.));
#85093=CARTESIAN_POINT('Ctrl Pts',(16.7454194590822,-19.6781104821466,-7.86510586795993));
#85094=CARTESIAN_POINT('Ctrl Pts',(16.7304230320966,-19.6370401442019,-7.86752224800844));
#85095=CARTESIAN_POINT('Ctrl Pts',(16.7166995414285,-19.5955068361058,-7.8699674126817));
#85096=CARTESIAN_POINT('Ctrl Pts',(16.6934926816934,-19.5172056306188,-7.8746296967584));
#85097=CARTESIAN_POINT('Ctrl Pts',(16.6836949864714,-19.4805607535186,-7.87683264517523));
#85098=CARTESIAN_POINT('Ctrl Pts',(16.6731275213978,-19.4363047058337,-7.87953975057152));
#85099=CARTESIAN_POINT('Ctrl Pts',(16.6714072156323,-19.4289249658938,-7.87999270481254));
#85100=CARTESIAN_POINT('Ctrl Pts',(16.6687987099737,-19.4174569087303,-7.8806992064329));
#85101=CARTESIAN_POINT('Ctrl Pts',(16.667882927276,-19.4133748403567,-7.88095119933021));
#85102=CARTESIAN_POINT('Ctrl Pts',(16.6662094742611,-19.4058105788483,-7.88141914790224));
#85103=CARTESIAN_POINT('Ctrl Pts',(16.6654484943428,-19.4023291770174,-7.88163491123376));
#85104=CARTESIAN_POINT('Ctrl Pts',(16.6637510201735,-19.3944683242684,-7.88212297776956));
#85105=CARTESIAN_POINT('Ctrl Pts',(16.6628196357975,-19.390087838844,-7.8823955674499));
#85106=CARTESIAN_POINT('Ctrl Pts',(16.660120228627,-19.3771909562168,-7.88319985232476));
#85107=CARTESIAN_POINT('Ctrl Pts',(16.6583908097984,-19.368666700081,-7.88373367139447));
#85108=CARTESIAN_POINT('Ctrl Pts',(16.6465062974476,-19.3081776448585,-7.88753627043884));
#85109=CARTESIAN_POINT('Ctrl Pts',(16.6382522153223,-19.255862929692,-7.89090069133754));
#85110=CARTESIAN_POINT('Ctrl Pts',(16.6301911620637,-19.1884349207003,-7.89528837021718));
#85111=CARTESIAN_POINT('Ctrl Pts',(16.6285718969084,-19.1735526702708,-7.89625999960626));
#85112=CARTESIAN_POINT('Ctrl Pts',(16.6204362928577,-19.0906084516964,-7.90168907697733));
#85113=CARTESIAN_POINT('Ctrl Pts',(16.6170625898356,-19.0222805698061,-7.90621169922116));
#85114=CARTESIAN_POINT('Ctrl Pts',(16.6168557120479,-18.7931414075279,-7.92135266217216));
#85115=CARTESIAN_POINT('Ctrl Pts',(16.6350247735661,-18.6328491686991,-7.93185066226681));
#85116=CARTESIAN_POINT('Ctrl Pts',(16.6765204031032,-18.4529688512325,-7.94322216467185));
#85117=CARTESIAN_POINT('Ctrl Pts',(16.6822553141319,-18.4298906288441,-7.94467444424136));
#85118=CARTESIAN_POINT('Ctrl Pts',(16.6908695970453,-18.3975626302714,-7.94670014317305));
#85119=CARTESIAN_POINT('Ctrl Pts',(16.6934253009823,-18.3882291750872,-7.94728396599734));
#85120=CARTESIAN_POINT('Ctrl Pts',(16.6976666647772,-18.3731464467184,-7.94822584779665));
#85121=CARTESIAN_POINT('Ctrl Pts',(16.6993128688492,-18.3673863089507,-7.94858518366482));
#85122=CARTESIAN_POINT('Ctrl Pts',(16.7027975180278,-18.3553863978649,-7.94933303086491));
#85123=CARTESIAN_POINT('Ctrl Pts',(16.7046403186936,-18.3491479465346,-7.94972139571439));
#85124=CARTESIAN_POINT('Ctrl Pts',(16.7090695324404,-18.3344041536795,-7.9506382951558));
#85125=CARTESIAN_POINT('Ctrl Pts',(16.7116808362905,-18.3259063715311,-7.95116600991541));
#85126=CARTESIAN_POINT('Ctrl Pts',(16.7205471826034,-18.2976875470883,-7.95291609207069));
#85127=CARTESIAN_POINT('Ctrl Pts',(16.7270379021795,-18.2780413836334,-7.95413072322058));
#85128=CARTESIAN_POINT('Ctrl Pts',(16.7631661561862,-18.1738417659314,-7.96055728524779));
#85129=CARTESIAN_POINT('Ctrl Pts',(16.7978624833675,-18.0911338970417,-7.96559779631823));
#85130=CARTESIAN_POINT('Ctrl Pts',(16.8976427994538,-17.8900855297674,-7.97797942744256));
#85131=CARTESIAN_POINT('Ctrl Pts',(16.9689850845162,-17.7753138247879,-7.98515787236621));
#85132=CARTESIAN_POINT('Ctrl Pts',(17.0971458320886,-17.607288592211,-7.99685013466944));
#85133=CARTESIAN_POINT('Ctrl Pts',(17.1467942734104,-17.5490332645751,-8.00116971420075));
#85134=CARTESIAN_POINT('Ctrl Pts',(17.2060220538967,-17.486714156302,-8.0062650856435));
#85135=CARTESIAN_POINT('Ctrl Pts',(17.2126111820274,-17.479873896548,-8.00683121545435));
#85136=CARTESIAN_POINT('Ctrl Pts',(17.22244624565,-17.4698005419395,-8.00767557491742));
#85137=CARTESIAN_POINT('Ctrl Pts',(17.2256571127177,-17.4665331645424,-8.00795113171247));
#85138=CARTESIAN_POINT('Ctrl Pts',(17.231390352827,-17.4607367748996,-8.00844303394105));
#85139=CARTESIAN_POINT('Ctrl Pts',(17.233908546069,-17.4582036993194,-8.008659050336));
#85140=CARTESIAN_POINT('Ctrl Pts',(17.2393381935503,-17.4527695385085,-8.00912474738892));
#85141=CARTESIAN_POINT('Ctrl Pts',(17.2422516463095,-17.4498705978107,-8.0093745836083));
#85142=CARTESIAN_POINT('Ctrl Pts',(17.2503213502874,-17.4418877200531,-8.01006639933602));
#85143=CARTESIAN_POINT('Ctrl Pts',(17.2554952156978,-17.436821781781,-8.010509750164));
#85144=CARTESIAN_POINT('Ctrl Pts',(17.284054844249,-17.4091434733207,-8.0129553924431));
#85145=CARTESIAN_POINT('Ctrl Pts',(17.3079320750152,-17.3870472144712,-8.01499401047398));
#85146=CARTESIAN_POINT('Ctrl Pts',(17.4542419685985,-17.2577796637008,-8.02739988205871));
#85147=CARTESIAN_POINT('Ctrl Pts',(17.588186180866,-17.1644671225473,-8.03835714537534));
#85148=CARTESIAN_POINT('Ctrl Pts',(17.8343783664717,-17.0321002963409,-8.05661523025183));
#85149=CARTESIAN_POINT('Ctrl Pts',(17.9416765750237,-16.9853873406102,-8.06405607123662));
#85150=CARTESIAN_POINT('Ctrl Pts',(18.0658261026039,-16.9431603278798,-8.07206312933223));
#85151=CARTESIAN_POINT('Ctrl Pts',(18.0794008224476,-16.9386959698272,-8.072931105485));
#85152=CARTESIAN_POINT('Ctrl Pts',(18.1010776394829,-16.9318094732524,-8.07430541422955));
#85153=CARTESIAN_POINT('Ctrl Pts',(18.1091506608241,-16.9292978999926,-8.07481467489004));
#85154=CARTESIAN_POINT('Ctrl Pts',(18.1234152326693,-16.9249536435684,-8.07571005311163));
#85155=CARTESIAN_POINT('Ctrl Pts',(18.1296004870851,-16.9231008109223,-8.0760968267999));
#85156=CARTESIAN_POINT('Ctrl Pts',(18.1424111095,-16.9193270878367,-8.07689489559987));
#85157=CARTESIAN_POINT('Ctrl Pts',(18.1490375905764,-16.9174102220598,-8.07730605533092));
#85158=CARTESIAN_POINT('Ctrl Pts',(18.1660708983198,-16.9125730308735,-8.07835876507018));
#85159=CARTESIAN_POINT('Ctrl Pts',(18.1764910164661,-16.9096999322398,-8.07899877377739));
#85160=CARTESIAN_POINT('Ctrl Pts',(18.2200727293667,-16.8980417234947,-8.0816594379043));
#85161=CARTESIAN_POINT('Ctrl Pts',(18.2534244813408,-16.8899832181597,-8.08365656461557));
#85162=CARTESIAN_POINT('Ctrl Pts',(18.3408211609655,-16.8711021270563,-8.08880063775893));
#85163=CARTESIAN_POINT('Ctrl Pts',(18.3951197442136,-16.8615726813116,-8.09190819529001));
#85164=CARTESIAN_POINT('Ctrl Pts',(18.558087537074,-16.8394895423993,-8.10105260331991));
#85165=CARTESIAN_POINT('Ctrl Pts',(18.6674213462009,-16.8332235147235,-8.10694072442736));
#85166=CARTESIAN_POINT('Ctrl Pts',(18.8224701916281,-16.8363551187521,-8.11538395477344));
#85167=CARTESIAN_POINT('Ctrl Pts',(18.8681477481271,-16.8387597432486,-8.11788438165609));
#85168=CARTESIAN_POINT('Ctrl Pts',(18.9364180536166,-16.8445761406398,-8.1216837269709));
#85169=CARTESIAN_POINT('Ctrl Pts',(18.9590926750583,-16.8468772892681,-8.12295598013379));
#85170=CARTESIAN_POINT('Ctrl Pts',(18.9827504056994,-16.8496647980315,-8.12429816534834));
#85171=CARTESIAN_POINT('Ctrl Pts',(18.9837755855149,-16.8497863518076,-8.12435635643155));
#85172=CARTESIAN_POINT('Ctrl Pts',(19.0030165219534,-16.8520819893648,-8.12544905957002));
#85173=CARTESIAN_POINT('Ctrl Pts',(19.0212028764875,-16.8544919516727,-8.12649116268315));
#85174=CARTESIAN_POINT('Ctrl Pts',(19.0724996166818,-16.8619691609641,-8.1294624883361));
#85175=CARTESIAN_POINT('Ctrl Pts',(19.1055227202059,-16.8675860572733,-8.13141308620021));
#85176=CARTESIAN_POINT('Ctrl Pts',(19.1451980358659,-16.8753071513822,-8.13381732359371));
#85177=CARTESIAN_POINT('Ctrl Pts',(19.1519928783091,-16.8766641325105,-8.13423123978184));
#85178=CARTESIAN_POINT('Ctrl Pts',(19.1631375823776,-16.8789467655288,-8.13491387024137));
#85179=CARTESIAN_POINT('Ctrl Pts',(19.1674914661766,-16.879852822437,-8.13518149102585));
#85180=CARTESIAN_POINT('Ctrl Pts',(19.1753272380623,-16.8815092476423,-8.13566487761919));
#85181=CARTESIAN_POINT('Ctrl Pts',(19.1788101114186,-16.8822546893133,-8.13588035953831));
#85182=CARTESIAN_POINT('Ctrl Pts',(19.18640402507,-16.8839000729682,-8.13635156049491));
#85183=CARTESIAN_POINT('Ctrl Pts',(19.1905142172713,-16.8848034735888,-8.13660747109534));
#85184=CARTESIAN_POINT('Ctrl Pts',(19.2021294427328,-16.8873927751305,-8.1373330825887));
#85185=CARTESIAN_POINT('Ctrl Pts',(19.2096279294223,-16.8891073133282,-8.13780437853594));
#85186=CARTESIAN_POINT('Ctrl Pts',(19.2560674190503,-16.8999924182554,-8.14074024373807));
#85187=CARTESIAN_POINT('Ctrl Pts',(19.2947486243764,-16.9102238107458,-8.143259982085));
#85188=CARTESIAN_POINT('Ctrl Pts',(19.4986171921126,-16.9703780099379,-8.15685569395482));
#85189=CARTESIAN_POINT('Ctrl Pts',(19.6575292055489,-17.0392628362193,-8.16850287167479));
#85190=CARTESIAN_POINT('Ctrl Pts',(19.8919426330622,-17.1769736794803,-8.18613287195658));
#85191=CARTESIAN_POINT('Ctrl Pts',(19.9739258016713,-17.2332392576233,-8.19241430282786));
#85192=CARTESIAN_POINT('Ctrl Pts',(20.0625882076603,-17.3037472530884,-8.19932817043001));
#85193=CARTESIAN_POINT('Ctrl Pts',(20.0734246214486,-17.3125411132536,-8.20017557044739));
#85194=CARTESIAN_POINT('Ctrl Pts',(20.0906103918501,-17.3267716814005,-8.20152353238014));
#85195=CARTESIAN_POINT('Ctrl Pts',(20.0970157400845,-17.3321398399048,-8.20202685024767));
#85196=CARTESIAN_POINT('Ctrl Pts',(20.1083013186278,-17.3417123318911,-8.20291533865471));
#85197=CARTESIAN_POINT('Ctrl Pts',(20.1131944332442,-17.3459012467546,-8.20330113353076));
#85198=CARTESIAN_POINT('Ctrl Pts',(20.1233191092686,-17.3546492042702,-8.20410063703401));
#85199=CARTESIAN_POINT('Ctrl Pts',(20.1285475322625,-17.3592117736433,-8.20451419318579));
#85200=CARTESIAN_POINT('Ctrl Pts',(20.1420024229867,-17.3710701857922,-8.20558029965285));
#85201=CARTESIAN_POINT('Ctrl Pts',(20.1501947191423,-17.3784046184098,-8.20623123097674));
#85202=CARTESIAN_POINT('Ctrl Pts',(20.1849394390229,-17.4100021266518,-8.20900020226171));
#85203=CARTESIAN_POINT('Ctrl Pts',(20.210929272352,-17.4348767857808,-8.21109219840875));
#85204=CARTESIAN_POINT('Ctrl Pts',(20.2777286433051,-17.5021542954613,-8.21653887715065));
#85205=CARTESIAN_POINT('Ctrl Pts',(20.3174268136529,-17.545617769574,-8.21984780785296));
#85206=CARTESIAN_POINT('Ctrl Pts',(20.4633879457798,-17.7194504503348,-8.23243226252002));
#85207=CARTESIAN_POINT('Ctrl Pts',(20.5557751105201,-17.8606297312796,-8.24128142180231));
#85208=CARTESIAN_POINT('Ctrl Pts',(20.6549175509313,-18.060491420903,-8.25381141611157));
#85209=CARTESIAN_POINT('Ctrl Pts',(20.677419578213,-18.1106730592126,-8.25696256627584));
#85210=CARTESIAN_POINT('Ctrl Pts',(20.7012202991938,-18.1698168744309,-8.26074538910701));
#85211=CARTESIAN_POINT('Ctrl Pts',(20.7044485520071,-18.1779853713692,-8.2612693404077));
#85212=CARTESIAN_POINT('Ctrl Pts',(20.7092525387811,-18.1903658166282,-8.26206605584896));
#85213=CARTESIAN_POINT('Ctrl Pts',(20.7108658822522,-18.1945632013353,-8.26233661824698));
#85214=CARTESIAN_POINT('Ctrl Pts',(20.7137342236981,-18.2020972649618,-8.26282312073175));
#85215=CARTESIAN_POINT('Ctrl Pts',(20.7149941770911,-18.2054320000536,-8.26303876014449));
#85216=CARTESIAN_POINT('Ctrl Pts',(20.7177095525902,-18.2126740933998,-8.26350773695192));
#85217=CARTESIAN_POINT('Ctrl Pts',(20.7191618364278,-18.2165825214845,-8.26376125184051));
#85218=CARTESIAN_POINT('Ctrl Pts',(20.7231986580862,-18.2275456210155,-8.26447347243599));
#85219=CARTESIAN_POINT('Ctrl Pts',(20.7257571703443,-18.2346097163639,-8.26493368272565));
#85220=CARTESIAN_POINT('Ctrl Pts',(20.7406307217082,-18.2763687755437,-8.26766115503635));
#85221=CARTESIAN_POINT('Ctrl Pts',(20.7520758182437,-18.3113643654059,-8.26997508052884));
#85222=CARTESIAN_POINT('Ctrl Pts',(20.7863631188612,-18.4262630177201,-8.27762383391845));
#85223=CARTESIAN_POINT('Ctrl Pts',(20.805414114031,-18.507212964824,-8.28309007395295));
#85224=CARTESIAN_POINT('Ctrl Pts',(20.850709648133,-18.7675115344248,-8.30054051516429));
#85225=CARTESIAN_POINT('Ctrl Pts',(20.8587385380537,-18.94924318391,-8.31245634036885));
#85226=CARTESIAN_POINT('Ctrl Pts',(20.8416283250973,-19.1522481744002,-8.32499026326175));
#85227=CARTESIAN_POINT('Ctrl Pts',(20.8393780671179,-19.1746650941409,-8.32636507902359));
#85228=CARTESIAN_POINT('Ctrl Pts',(20.8356742486542,-19.2064484738305,-8.32830184130312));
#85229=CARTESIAN_POINT('Ctrl Pts',(20.8345150314787,-19.2158470776419,-8.32887300444326));
#85230=CARTESIAN_POINT('Ctrl Pts',(20.8325244310284,-19.2311409152854,-8.32979997686675));
#85231=CARTESIAN_POINT('Ctrl Pts',(20.8317311848015,-19.2370409017061,-8.33015698515062));
#85232=CARTESIAN_POINT('Ctrl Pts',(20.8300146874149,-19.2494124442066,-8.33090436845387));
#85233=CARTESIAN_POINT('Ctrl Pts',(20.8290863255787,-19.2558832369165,-8.3312945777079));
#85234=CARTESIAN_POINT('Ctrl Pts',(20.8267986896732,-19.2713193809645,-8.3322238012155));
#85235=CARTESIAN_POINT('Ctrl Pts',(20.825411749673,-19.2802805504172,-8.3327619340338));
#85236=CARTESIAN_POINT('Ctrl Pts',(20.8205047426559,-19.3106912604255,-8.33458389999213));
#85237=CARTESIAN_POINT('Ctrl Pts',(20.8167118538631,-19.3320958391715,-8.33585908360513));
#85238=CARTESIAN_POINT('Ctrl Pts',(20.7939488841615,-19.4499590775858,-8.34284659366596));
#85239=CARTESIAN_POINT('Ctrl Pts',(20.7686067000857,-19.5450695713826,-8.34835040425284));
#85240=CARTESIAN_POINT('Ctrl Pts',(20.6933418744,-19.764774663746,-8.36110828161006));
#85241=CARTESIAN_POINT('Ctrl Pts',(20.6380203207323,-19.8870544231139,-8.36823789870716));
#85242=CARTESIAN_POINT('Ctrl Pts',(20.5637979768948,-20.0167865345906,-8.37655430229737));
#85243=CARTESIAN_POINT('Ctrl Pts',(20.555924355507,-20.0302034253452,-8.37742421158511));
#85244=CARTESIAN_POINT('Ctrl Pts',(20.5207030926731,-20.0887339815106,-8.38126781467058));
#85245=CARTESIAN_POINT('Ctrl Pts',(20.4918246986183,-20.1328994140527,-8.3842962425026));
#85246=CARTESIAN_POINT('Ctrl Pts',(20.4563044996808,-20.1830287443011,-8.38794236120464));
#85247=CARTESIAN_POINT('Ctrl Pts',(20.4512354442606,-20.1900900540865,-8.38846095849569));
#85248=CARTESIAN_POINT('Ctrl Pts',(20.4434898382314,-20.2007407812396,-8.38925110646511));
#85249=CARTESIAN_POINT('Ctrl Pts',(20.4408450791874,-20.2043533529137,-8.38952050920648));
#85250=CARTESIAN_POINT('Ctrl Pts',(20.43607472904,-20.2108261658927,-8.39000577717004));
#85251=CARTESIAN_POINT('Ctrl Pts',(20.4339533600845,-20.2136894516517,-8.39022134832604));
#85252=CARTESIAN_POINT('Ctrl Pts',(20.4293252254273,-20.2199033441032,-8.39069117404181));
#85253=CARTESIAN_POINT('Ctrl Pts',(20.4268157846041,-20.2232518352607,-8.3909456115316));
#85254=CARTESIAN_POINT('Ctrl Pts',(20.4197315604927,-20.23264655225,-8.39166297885597));
#85255=CARTESIAN_POINT('Ctrl Pts',(20.4151342531794,-20.2386756019387,-8.39212744776092));
#85256=CARTESIAN_POINT('Ctrl Pts',(20.3872994415457,-20.2747751808865,-8.39493258803806));
#85257=CARTESIAN_POINT('Ctrl Pts',(20.3632895852967,-20.3042382388064,-8.397323007135));
#85258=CARTESIAN_POINT('Ctrl Pts',(20.2812806025722,-20.3995170425488,-8.40535036437698));
#85259=CARTESIAN_POINT('Ctrl Pts',(20.2199865612467,-20.4623724231942,-8.41113225867746));
#85260=CARTESIAN_POINT('Ctrl Pts',(20.0256724758027,-20.6383272958077,-8.42845298969269));
#85261=CARTESIAN_POINT('Ctrl Pts',(19.8823664736713,-20.739007284665,-8.43990126181429));
#85262=CARTESIAN_POINT('Ctrl Pts',(19.7079463363748,-20.8318003800597,-8.45206277430418));
#85263=CARTESIAN_POINT('Ctrl Pts',(19.687408551335,-20.8422997474715,-8.45347080028325));
#85264=CARTESIAN_POINT('Ctrl Pts',(19.6581222052432,-20.8566728082937,-8.45544567752015));
#85265=CARTESIAN_POINT('Ctrl Pts',(19.6495132501926,-20.8608257778764,-8.45602224648443));
#85266=CARTESIAN_POINT('Ctrl Pts',(19.6354827951028,-20.8674773292086,-8.45695557845937));
#85267=CARTESIAN_POINT('Ctrl Pts',(19.6300784055993,-20.8700115017202,-8.45731357354201));
#85268=CARTESIAN_POINT('Ctrl Pts',(19.6187460598519,-20.8752670002481,-8.45806111135696));
#85269=CARTESIAN_POINT('Ctrl Pts',(19.6128160914703,-20.8779838585793,-8.45845049670276));
#85270=CARTESIAN_POINT('Ctrl Pts',(19.5986839755579,-20.8843797324103,-8.45937428110823));
#85271=CARTESIAN_POINT('Ctrl Pts',(19.5904707227049,-20.888034016427,-8.45990782597413));
#85272=CARTESIAN_POINT('Ctrl Pts',(19.562745838934,-20.9001585591861,-8.4616978768979));
#85273=CARTESIAN_POINT('Ctrl Pts',(19.543129496357,-20.9083872172852,-8.46294614564272));
#85274=CARTESIAN_POINT('Ctrl Pts',(19.3794566472617,-20.9741616773173,-8.47321885831932));
#85275=CARTESIAN_POINT('Ctrl Pts',(19.2295971413606,-21.0160114061446,-8.4816693188242));
#85276=CARTESIAN_POINT('Ctrl Pts',(18.9422190217862,-21.0631248601586,-8.49748366779995));
#85277=CARTESIAN_POINT('Ctrl Pts',(18.8061526482159,-21.0721384587118,-8.50483421515098));
#85278=CARTESIAN_POINT('Ctrl Pts',(18.6545760401514,-21.0675672259243,-8.51372642082399));
#85279=CARTESIAN_POINT('Ctrl Pts',(18.6389735479622,-21.0669238270284,-8.51465023432401));
#85280=CARTESIAN_POINT('Ctrl Pts',(18.6176090194386,-21.0658059363226,-8.51592859162525));
#85281=CARTESIAN_POINT('Ctrl Pts',(18.6118392565018,-21.0654803400444,-8.5162751664776));
#85282=CARTESIAN_POINT('Ctrl Pts',(18.602668315446,-21.0649251309896,-8.51682827134775));
#85283=CARTESIAN_POINT('Ctrl Pts',(18.5992661850041,-21.0647109171044,-8.51703394403361));
#85284=CARTESIAN_POINT('Ctrl Pts',(18.5922369100759,-21.0642512736052,-8.51745992859139));
#85285=CARTESIAN_POINT('Ctrl Pts',(18.5886098860117,-21.0640047183867,-8.51768030527992));
#85286=CARTESIAN_POINT('Ctrl Pts',(18.5799624978535,-21.0633945118143,-8.51820706103952));
#85287=CARTESIAN_POINT('Ctrl Pts',(18.5749427762321,-21.0630222961763,-8.51851391660689));
#85288=CARTESIAN_POINT('Ctrl Pts',(18.5579880449292,-21.0617042758174,-8.51955389670345));
#85289=CARTESIAN_POINT('Ctrl Pts',(18.5460599999924,-21.0606751482702,-8.52029147151354));
#85290=CARTESIAN_POINT('Ctrl Pts',(18.4091264926598,-21.0476897523819,-8.52882196998391));
#85291=CARTESIAN_POINT('Ctrl Pts',(18.2854270831029,-21.0247358854845,-8.53711883960778));
#85292=CARTESIAN_POINT('Ctrl Pts',(18.0034837829291,-20.9459874005889,-8.55646409421056));
#85293=CARTESIAN_POINT('Ctrl Pts',(17.848325523587,-20.8820882964693,-8.56740717984012));
#85294=CARTESIAN_POINT('Ctrl Pts',(17.681779601747,-20.7891370909323,-8.5791527797003));
#85295=CARTESIAN_POINT('Ctrl Pts',(17.6614651719961,-20.7773519030031,-8.58058682556847));
#85296=CARTESIAN_POINT('Ctrl Pts',(17.6332581851248,-20.76035442301,-8.5825807005051));
#85297=CARTESIAN_POINT('Ctrl Pts',(17.6251986285184,-20.7554239061748,-8.58315072412566));
#85298=CARTESIAN_POINT('Ctrl Pts',(17.6116111713855,-20.7469861194556,-8.58411233619252));
#85299=CARTESIAN_POINT('Ctrl Pts',(17.6060660970866,-20.7435068975004,-8.58450494908714));
#85300=CARTESIAN_POINT('Ctrl Pts',(17.5951046719161,-20.7365581537137,-8.58528144952721));
#85301=CARTESIAN_POINT('Ctrl Pts',(17.5896878206877,-20.7330895569855,-8.58566536572776));
#85302=CARTESIAN_POINT('Ctrl Pts',(17.5788372269676,-20.7260716133255,-8.58643481778078));
#85303=CARTESIAN_POINT('Ctrl Pts',(17.5734038300919,-20.7225218590102,-8.58682033293355));
#85304=CARTESIAN_POINT('Ctrl Pts',(17.5541553609242,-20.7098197421021,-8.58818691204402));
#85305=CARTESIAN_POINT('Ctrl Pts',(17.5404312927251,-20.7005300633227,-8.58916282533725));
#85306=CARTESIAN_POINT('Ctrl Pts',(17.422939699676,-20.6189732603783,-8.59753479661582));
#85307=CARTESIAN_POINT('Ctrl Pts',(17.3257253134569,-20.5377009495113,-8.6045571525512));
#85308=CARTESIAN_POINT('Ctrl Pts',(17.1406295607827,-20.3524273884892,-8.61884914417775));
#85309=CARTESIAN_POINT('Ctrl Pts',(17.0543431584248,-20.2476749032565,-8.62607107852499));
#85310=CARTESIAN_POINT('Ctrl Pts',(16.95247570486,-20.0965758266773,-8.63637781747498));
#85311=CARTESIAN_POINT('Ctrl Pts',(16.9275921294496,-20.056885753053,-8.63907800668033));
#85312=CARTESIAN_POINT('Ctrl Pts',(16.9001864898759,-20.009769336389,-8.64231459582629));
#85313=CARTESIAN_POINT('Ctrl Pts',(16.8963620362606,-20.0031111592495,-8.64277267689436));
#85314=CARTESIAN_POINT('Ctrl Pts',(16.8902925899454,-19.9924101927577,-8.64351027281511));
#85315=CARTESIAN_POINT('Ctrl Pts',(16.8880244351529,-19.9883805267096,-8.64378833912235));
#85316=CARTESIAN_POINT('Ctrl Pts',(16.8840211912224,-19.9812134186804,-8.64428351098323));
#85317=CARTESIAN_POINT('Ctrl Pts',(16.8822808489924,-19.9780789636951,-8.64450027573602));
#85318=CARTESIAN_POINT('Ctrl Pts',(16.8785983976439,-19.9714067788319,-8.64496215324987));
#85319=CARTESIAN_POINT('Ctrl Pts',(16.8766584699706,-19.9678679672834,-8.64520739347619));
#85320=CARTESIAN_POINT('Ctrl Pts',(16.8714269530806,-19.958259568714,-8.6458739381007));
#85321=CARTESIAN_POINT('Ctrl Pts',(16.8681549539663,-19.9521794518461,-8.64629645632944));
#85322=CARTESIAN_POINT('Ctrl Pts',(16.8517661886613,-19.9213651085607,-8.64844108093734));
#85323=CARTESIAN_POINT('Ctrl Pts',(16.8391119302808,-19.896389676674,-8.65018994855127));
#85324=CARTESIAN_POINT('Ctrl Pts',(16.8035648371587,-19.8226387218721,-8.6553692384259));
#85325=CARTESIAN_POINT('Ctrl Pts',(16.7820350890976,-19.7732331571053,-8.65885725237295));
#85326=CARTESIAN_POINT('Ctrl Pts',(16.7565777928111,-19.7081396808811,-8.663431461056));
#85327=CARTESIAN_POINT('Ctrl Pts',(16.7509125212525,-19.6931541927726,-8.66448311665522));
#85328=CARTESIAN_POINT('Ctrl Pts',(16.7454194712032,-19.678110515342,-8.66553666923996));
#85329=CARTESIAN_POINT('',(16.6172480955499,-18.9524633046122,-7.68905625083761));
#85330=CARTESIAN_POINT('Ctrl Pts',(16.7454194499637,-19.6781104571739,-8.4444886490522));
#85331=CARTESIAN_POINT('Ctrl Pts',(16.7701773775376,-19.7459143742589,-8.44016252692827));
#85332=CARTESIAN_POINT('Ctrl Pts',(16.798398965251,-19.8124279737233,-8.43583640480434));
#85333=CARTESIAN_POINT('Ctrl Pts',(16.8299125176285,-19.877278260566,-8.43151028268041));
#85334=CARTESIAN_POINT('Ctrl Pts',(16.8614397440995,-19.9421566866955,-8.42718228340223));
#85335=CARTESIAN_POINT('Ctrl Pts',(16.8962615401651,-20.0053699294018,-8.42285428412405));
#85336=CARTESIAN_POINT('Ctrl Pts',(16.9341606764734,-20.0665705044936,-8.41852628484587));
#85337=CARTESIAN_POINT('Ctrl Pts',(16.9721294353055,-20.1278835079655,-8.41419033482626));
#85338=CARTESIAN_POINT('Ctrl Pts',(17.0131865446795,-20.1871760506629,-8.40985438480666));
#85339=CARTESIAN_POINT('Ctrl Pts',(17.057072299101,-20.2441309863778,-8.40551843478705));
#85340=CARTESIAN_POINT('Ctrl Pts',(17.0972716608073,-20.2963017213222,-8.40154670351625));
#85341=CARTESIAN_POINT('Ctrl Pts',(17.1398437332676,-20.3465112515435,-8.39757497224546));
#85342=CARTESIAN_POINT('Ctrl Pts',(17.1845622179524,-20.3945434342034,-8.39360324097466));
#85343=CARTESIAN_POINT('Ctrl Pts',(17.2339699045481,-20.447612294745,-8.38921503204376));
#85344=CARTESIAN_POINT('Ctrl Pts',(17.2862036327227,-20.4982434590661,-8.38482682311286));
#85345=CARTESIAN_POINT('Ctrl Pts',(17.3409933109755,-20.5461208750697,-8.38043861418196));
#85346=CARTESIAN_POINT('Ctrl Pts',(17.3957016722616,-20.5939272330498,-8.37605691808069));
#85347=CARTESIAN_POINT('Ctrl Pts',(17.4529580928701,-20.6389876412174,-8.37167522197941));
#85348=CARTESIAN_POINT('Ctrl Pts',(17.5124544762694,-20.6810215537852,-8.36729352587814));
#85349=CARTESIAN_POINT('Ctrl Pts',(17.5718809466833,-20.7230060731605,-8.3629169786185));
#85350=CARTESIAN_POINT('Ctrl Pts',(17.6335417591178,-20.7619708847355,-8.35854043135886));
#85351=CARTESIAN_POINT('Ctrl Pts',(17.6970957742217,-20.7976756558407,-8.35416388409922));
#85352=CARTESIAN_POINT('Ctrl Pts',(17.7606094842929,-20.8333577834991,-8.34979011238225));
#85353=CARTESIAN_POINT('Ctrl Pts',(17.8260135952853,-20.8657837371302,-8.34541634066528));
#85354=CARTESIAN_POINT('Ctrl Pts',(17.8929392167478,-20.8947572568067,-8.34104256894831));
#85355=CARTESIAN_POINT('Ctrl Pts',(17.9598444725189,-20.923721959744,-8.33667012818475));
#85356=CARTESIAN_POINT('Ctrl Pts',(18.028269877152,-20.949236122938,-8.33229768742119));
#85357=CARTESIAN_POINT('Ctrl Pts',(18.097824766941,-20.9711508296416,-8.32792524665764));
#85358=CARTESIAN_POINT('Ctrl Pts',(18.1673814352561,-20.9930660967066,-8.32355269409029));
#85359=CARTESIAN_POINT('Ctrl Pts',(18.238067185385,-21.0113815814964,-8.31918014152294));
#85360=CARTESIAN_POINT('Ctrl Pts',(18.3094759435902,-21.0259981498375,-8.31480758895559));
#85361=CARTESIAN_POINT('Ctrl Pts',(18.3809588124981,-21.0406298878046,-8.31043049838827));
#85362=CARTESIAN_POINT('Ctrl Pts',(18.4531657140464,-21.0515549478117,-8.30605340782094));
#85363=CARTESIAN_POINT('Ctrl Pts',(18.5256809453891,-21.0587254618213,-8.30167631725361));
#85364=CARTESIAN_POINT('Ctrl Pts',(18.5982357799911,-21.0658998919146,-8.29729683619467));
#85365=CARTESIAN_POINT('Ctrl Pts',(18.6710987974685,-21.0693156708867,-8.29291735513573));
#85366=CARTESIAN_POINT('Ctrl Pts',(18.7438524696364,-21.0689770732916,-8.28853787407679));
#85367=CARTESIAN_POINT('Ctrl Pts',(18.8167350971998,-21.0686378755345,-8.28415063041707));
#85368=CARTESIAN_POINT('Ctrl Pts',(18.8895075103798,-21.064531039433,-8.27976338675735));
#85369=CARTESIAN_POINT('Ctrl Pts',(18.9617560690986,-21.0567128481075,-8.27537614309762));
#85370=CARTESIAN_POINT('Ctrl Pts',(19.0108781271724,-21.0513972313653,-8.27239324016283));
#85371=CARTESIAN_POINT('Ctrl Pts',(19.0597581560645,-21.0443670563134,-8.26941033722803));
#85372=CARTESIAN_POINT('Ctrl Pts',(19.1082694567067,-21.0356533717911,-8.26642743429324));
#85373=CARTESIAN_POINT('Ctrl Pts',(19.1796354137561,-21.0228344939807,-8.26203922536235));
#85374=CARTESIAN_POINT('Ctrl Pts',(19.2504813367645,-21.0063198837036,-8.25765101643146));
#85375=CARTESIAN_POINT('Ctrl Pts',(19.3203952805279,-20.9861655721633,-8.25326280750057));
#85376=CARTESIAN_POINT('Ctrl Pts',(19.3902054604071,-20.9660411729629,-8.24888111139929));
#85377=CARTESIAN_POINT('Ctrl Pts',(19.4590859472334,-20.9422879285591,-8.24449941529801));
#85378=CARTESIAN_POINT('Ctrl Pts',(19.526634079588,-20.9150130452637,-8.24011771919673));
#85379=CARTESIAN_POINT('Ctrl Pts',(19.5941028375112,-20.887770212127,-8.23574117193709));
#85380=CARTESIAN_POINT('Ctrl Pts',(19.6602419060116,-20.8570141403841,-8.23136462467746));
#85381=CARTESIAN_POINT('Ctrl Pts',(19.724664551087,-20.8229015867275,-8.22698807741782));
#85382=CARTESIAN_POINT('Ctrl Pts',(19.7890463402572,-20.7888106667567,-8.22261430570085));
#85383=CARTESIAN_POINT('Ctrl Pts',(19.8517134405357,-20.7513677135307,-8.21824053398388));
#85384=CARTESIAN_POINT('Ctrl Pts',(19.9123011549775,-20.7107766737647,-8.21386676226691));
#85385=CARTESIAN_POINT('Ctrl Pts',(19.9728704323744,-20.6701979859884,-8.20949432150336));
#85386=CARTESIAN_POINT('Ctrl Pts',(20.0313611796541,-20.6264733818696,-8.20512188073982));
#85387=CARTESIAN_POINT('Ctrl Pts',(20.0874367225441,-20.5798507419506,-8.20074943997627));
#85388=CARTESIAN_POINT('Ctrl Pts',(20.1435136992921,-20.5332269098853,-8.19637688740892));
#85389=CARTESIAN_POINT('Ctrl Pts',(20.1971749793955,-20.4837052048255,-8.19200433484156));
#85390=CARTESIAN_POINT('Ctrl Pts',(20.2481174066906,-20.4315734110738,-8.18763178227421));
#85391=CARTESIAN_POINT('Ctrl Pts',(20.2991127039582,-20.3793875129803,-8.18325469170688));
#85392=CARTESIAN_POINT('Ctrl Pts',(20.3473831767919,-20.3245864635399,-8.17887760113956));
#85393=CARTESIAN_POINT('Ctrl Pts',(20.3926635636811,-20.2674938929986,-8.17450051057223));
#85394=CARTESIAN_POINT('Ctrl Pts',(20.4379686798702,-20.2103701420857,-8.17012102951329));
#85395=CARTESIAN_POINT('Ctrl Pts',(20.4802801788311,-20.1509527715819,-8.16574154845435));
#85396=CARTESIAN_POINT('Ctrl Pts',(20.5193756546998,-20.0895951703508,-8.16136206739541));
#85397=CARTESIAN_POINT('Ctrl Pts',(20.558540427037,-20.0281288131833,-8.15697482373569));
#85398=CARTESIAN_POINT('Ctrl Pts',(20.594477554813,-19.9647157776937,-8.15258758007597));
#85399=CARTESIAN_POINT('Ctrl Pts',(20.627010467696,-19.8997343347128,-8.14820033641625));
#85400=CARTESIAN_POINT('Ctrl Pts',(20.6491297135924,-19.8555532150827,-8.14521743348143));
#85401=CARTESIAN_POINT('Ctrl Pts',(20.6696762814795,-19.8106475457985,-8.14223453054661));
#85402=CARTESIAN_POINT('Ctrl Pts',(20.6886076987149,-19.7651406668741,-8.1392516276118));
#85403=CARTESIAN_POINT('Ctrl Pts',(20.7164580900962,-19.6981945754734,-8.1348634186809));
#85404=CARTESIAN_POINT('Ctrl Pts',(20.7409194707722,-19.6296853205151,-8.13047520975));
#85405=CARTESIAN_POINT('Ctrl Pts',(20.7618159759921,-19.5599896113515,-8.1260870008191));
#85406=CARTESIAN_POINT('Ctrl Pts',(20.7826814673335,-19.4903973421759,-8.12170530471784));
#85407=CARTESIAN_POINT('Ctrl Pts',(20.7999924489196,-19.4196225726486,-8.11732360861657));
#85408=CARTESIAN_POINT('Ctrl Pts',(20.813621111304,-19.3480619060435,-8.1129419125153));
#85409=CARTESIAN_POINT('Ctrl Pts',(20.8272337589254,-19.2765853289167,-8.10856536525566));
#85410=CARTESIAN_POINT('Ctrl Pts',(20.8371725931962,-19.204325160743,-8.10418881799602));
#85411=CARTESIAN_POINT('Ctrl Pts',(20.8433600899069,-19.1316914330405,-8.09981227073638));
#85412=CARTESIAN_POINT('Ctrl Pts',(20.849543662597,-19.0591037685925,-8.09543849901941));
#85413=CARTESIAN_POINT('Ctrl Pts',(20.8519805772149,-18.9861434941225,-8.09106472730244));
#85414=CARTESIAN_POINT('Ctrl Pts',(20.8506449171335,-18.9132276545351,-8.08669095558547));
#85415=CARTESIAN_POINT('Ctrl Pts',(20.849309663498,-18.8403340034827,-8.08231851482192));
#85416=CARTESIAN_POINT('Ctrl Pts',(20.8442041231405,-18.7674852424751,-8.07794607405836));
#85417=CARTESIAN_POINT('Ctrl Pts',(20.8353544889708,-18.6950986343318,-8.07357363329482));
#85418=CARTESIAN_POINT('Ctrl Pts',(20.826504628515,-18.6227101752547,-8.06920108072747));
#85419=CARTESIAN_POINT('Ctrl Pts',(20.8139105446927,-18.550784371074,-8.06482852816012));
#85420=CARTESIAN_POINT('Ctrl Pts',(20.7976501258781,-18.4797319003326,-8.06045597559277));
#85421=CARTESIAN_POINT('Ctrl Pts',(20.7813728313875,-18.4086056886572,-8.05607888502545));
#85422=CARTESIAN_POINT('Ctrl Pts',(20.7614217126851,-18.338355091294,-8.05170179445812));
#85423=CARTESIAN_POINT('Ctrl Pts',(20.7379253105678,-18.2693783261091,-8.0473247038908));
#85424=CARTESIAN_POINT('Ctrl Pts',(20.7144160761932,-18.2003638901525,-8.04294522283186));
#85425=CARTESIAN_POINT('Ctrl Pts',(20.6873578824888,-18.1326251197522,-8.03856574177292));
#85426=CARTESIAN_POINT('Ctrl Pts',(20.6569274894877,-18.0665403057323,-8.03418626071398));
#85427=CARTESIAN_POINT('Ctrl Pts',(20.6264431588193,-18.0003383568232,-8.02979901705427));
#85428=CARTESIAN_POINT('Ctrl Pts',(20.5925749169665,-17.9357966461503,-8.02541177339455));
#85429=CARTESIAN_POINT('Ctrl Pts',(20.555545255664,-17.8732683922458,-8.02102452973483));
#85430=CARTESIAN_POINT('Ctrl Pts',(20.5303686541479,-17.8307552047989,-8.01804162680001));
#85431=CARTESIAN_POINT('Ctrl Pts',(20.5037315602569,-17.7891722056905,-8.01505872386519));
#85432=CARTESIAN_POINT('Ctrl Pts',(20.475714693788,-17.7486218693016,-8.01207582093037));
#85433=CARTESIAN_POINT('Ctrl Pts',(20.4344985139989,-17.6889674480277,-8.00768761199947));
#85434=CARTESIAN_POINT('Ctrl Pts',(20.3901335538166,-17.6313165376484,-8.00329940306857));
#85435=CARTESIAN_POINT('Ctrl Pts',(20.342841373937,-17.5760209182155,-7.99891119413767));
#85436=CARTESIAN_POINT('Ctrl Pts',(20.2956193834937,-17.5208073666502,-7.99452949803641));
#85437=CARTESIAN_POINT('Ctrl Pts',(20.2454791086752,-17.4679425302631,-7.99014780193516));
#85438=CARTESIAN_POINT('Ctrl Pts',(20.1926848492421,-17.4177485504026,-7.9857661058339));
#85439=CARTESIAN_POINT('Ctrl Pts',(20.1399526272652,-17.367613552463,-7.98138955857425));
#85440=CARTESIAN_POINT('Ctrl Pts',(20.0845729637365,-17.3201435071859,-7.97701301131462));
#85441=CARTESIAN_POINT('Ctrl Pts',(20.0268486678897,-17.2756255424471,-7.97263646405497));
#85442=CARTESIAN_POINT('Ctrl Pts',(19.9691609799523,-17.2311358103545,-7.968262692338));
#85443=CARTESIAN_POINT('Ctrl Pts',(19.9091319909997,-17.1895947380413,-7.96388892062103));
#85444=CARTESIAN_POINT('Ctrl Pts',(19.8470983416193,-17.1512498557866,-7.95951514890405));
#85445=CARTESIAN_POINT('Ctrl Pts',(19.7850835692867,-17.1129166420084,-7.9551427081405));
#85446=CARTESIAN_POINT('Ctrl Pts',(19.7210657576844,-17.0777779408324,-7.95077026737695));
#85447=CARTESIAN_POINT('Ctrl Pts',(19.6554099365354,-17.0460375846167,-7.9463978266134));
#85448=CARTESIAN_POINT('Ctrl Pts',(19.5897524365599,-17.0142964167966,-7.94202527404605));
#85449=CARTESIAN_POINT('Ctrl Pts',(19.5224572790419,-16.9859539746119,-7.9376527214787));
#85450=CARTESIAN_POINT('Ctrl Pts',(19.4539119391446,-16.9611670587724,-7.93328016891136));
#85451=CARTESIAN_POINT('Ctrl Pts',(19.385295460308,-16.9363544181366,-7.92890307834403));
#85452=CARTESIAN_POINT('Ctrl Pts',(19.3154266631729,-16.9151048356875,-7.9245259877767));
#85453=CARTESIAN_POINT('Ctrl Pts',(19.2447099626404,-16.8975257767351,-7.92014889720936));
#85454=CARTESIAN_POINT('Ctrl Pts',(19.1739546410931,-16.8799371172062,-7.91576941615042));
#85455=CARTESIAN_POINT('Ctrl Pts',(19.1023509680262,-16.8660230644093,-7.91138993509147));
#85456=CARTESIAN_POINT('Ctrl Pts',(19.0303127030105,-16.8558397527778,-7.90701045403253));
#85457=CARTESIAN_POINT('Ctrl Pts',(18.9581467506537,-16.8456383912948,-7.90262321037281));
#85458=CARTESIAN_POINT('Ctrl Pts',(18.8855451489719,-16.8391810190706,-7.89823596671308));
#85459=CARTESIAN_POINT('Ctrl Pts',(18.8129253294089,-16.8364717462587,-7.89384872305336));
#85460=CARTESIAN_POINT('Ctrl Pts',(18.7635508497353,-16.8346297018115,-7.89086582011855));
#85461=CARTESIAN_POINT('Ctrl Pts',(18.7141679744269,-16.834519193629,-7.88788291718374));
#85462=CARTESIAN_POINT('Ctrl Pts',(18.6649065603161,-16.8361278165748,-7.88490001424893));
#85463=CARTESIAN_POINT('Ctrl Pts',(18.5924370961486,-16.8384942943756,-7.88051180531803));
#85464=CARTESIAN_POINT('Ctrl Pts',(18.5199478924754,-16.8445928606293,-7.87612359638714));
#85465=CARTESIAN_POINT('Ctrl Pts',(18.4478546672522,-16.8544276297237,-7.87173538745625));
#85466=CARTESIAN_POINT('Ctrl Pts',(18.3758684403285,-16.8642478023901,-7.86735369135498));
#85467=CARTESIAN_POINT('Ctrl Pts',(18.3042774991949,-16.8777931053665,-7.86297199525372));
#85468=CARTESIAN_POINT('Ctrl Pts',(18.2334957741929,-16.8950156733827,-7.85859029915245));
#85469=CARTESIAN_POINT('Ctrl Pts',(18.1627972233507,-16.9122180035109,-7.85421375189281));
#85470=CARTESIAN_POINT('Ctrl Pts',(18.0929064660606,-16.9330889013489,-7.84983720463317));
#85471=CARTESIAN_POINT('Ctrl Pts',(18.0242288363219,-16.957529169125,-7.84546065737353));
#85472=CARTESIAN_POINT('Ctrl Pts',(17.9555947609379,-16.9819539372385,-7.84108688565657));
#85473=CARTESIAN_POINT('Ctrl Pts',(17.8881727399597,-17.0099434225998,-7.8367131139396));
#85474=CARTESIAN_POINT('Ctrl Pts',(17.8223531243443,-17.0413485471946,-7.83233934222264));
#85475=CARTESIAN_POINT('Ctrl Pts',(17.7565535378591,-17.0727441151046,-7.82796690145909));
#85476=CARTESIAN_POINT('Ctrl Pts',(17.6923558237636,-17.1075530511353,-7.82359446069555));
#85477=CARTESIAN_POINT('Ctrl Pts',(17.6301289564798,-17.1455787536464,-7.819222019932));
#85478=CARTESIAN_POINT('Ctrl Pts',(17.5679004980477,-17.1836054284792,-7.81484946736464));
#85479=CARTESIAN_POINT('Ctrl Pts',(17.5076433970481,-17.2248487798647,-7.81047691479728));
#85480=CARTESIAN_POINT('Ctrl Pts',(17.4496992310201,-17.2690678757604,-7.80610436222991));
#85481=CARTESIAN_POINT('Ctrl Pts',(17.3916949283513,-17.3133328639015,-7.80172727166259));
#85482=CARTESIAN_POINT('Ctrl Pts',(17.3360087376083,-17.3605794693657,-7.79735018109527));
#85483=CARTESIAN_POINT('Ctrl Pts',(17.2829499222259,-17.4105258121552,-7.79297309052795));
#85484=CARTESIAN_POINT('Ctrl Pts',(17.2298621294551,-17.4604994324963,-7.78859360946901));
#85485=CARTESIAN_POINT('Ctrl Pts',(17.1794049028396,-17.5131753771404,-7.78421412841008));
#85486=CARTESIAN_POINT('Ctrl Pts',(17.1318494027623,-17.5682361242716,-7.77983464735114));
#85487=CARTESIAN_POINT('Ctrl Pts',(17.0842096108804,-17.6233944662074,-7.77544740369142));
#85488=CARTESIAN_POINT('Ctrl Pts',(17.0394821127491,-17.6809456706579,-7.7710601600317));
#85489=CARTESIAN_POINT('Ctrl Pts',(16.9978963120804,-17.7405409685871,-7.76667291637198));
#85490=CARTESIAN_POINT('Ctrl Pts',(16.9696219748237,-17.7810600285899,-7.76369001343715));
#85491=CARTESIAN_POINT('Ctrl Pts',(16.9427990411462,-17.8225233957318,-7.76070711050233));
#85492=CARTESIAN_POINT('Ctrl Pts',(16.9174873693318,-17.864815166302,-7.7577242075675));
#85493=CARTESIAN_POINT('Ctrl Pts',(16.8789674908493,-17.9291757456869,-7.75318475796428));
#85494=CARTESIAN_POINT('Ctrl Pts',(16.843807884674,-17.995692576386,-7.74864530836106));
#85495=CARTESIAN_POINT('Ctrl Pts',(16.8122472000427,-18.0639937073104,-7.74410585875784));
#85496=CARTESIAN_POINT('Ctrl Pts',(16.7803526868129,-18.1330172836152,-7.73951839377989));
#85497=CARTESIAN_POINT('Ctrl Pts',(16.7521339850622,-18.2038627902841,-7.73493092880195));
#85498=CARTESIAN_POINT('Ctrl Pts',(16.727791895044,-18.2761168447069,-7.730343463824));
#85499=CARTESIAN_POINT('Ctrl Pts',(16.7037989805433,-18.3473344496374,-7.72582180381417));
#85500=CARTESIAN_POINT('Ctrl Pts',(16.6835723608134,-18.4199200369919,-7.72130014380433));
#85501=CARTESIAN_POINT('Ctrl Pts',(16.6672572513858,-18.493455115555,-7.7167784837945));
#85502=CARTESIAN_POINT('Ctrl Pts',(16.6505859845116,-18.5685954586082,-7.7121581163325));
#85503=CARTESIAN_POINT('Ctrl Pts',(16.6379992287984,-18.6447268210055,-7.7075377488705));
#85504=CARTESIAN_POINT('Ctrl Pts',(16.6295984951253,-18.7213849391715,-7.7029173814085));
#85505=CARTESIAN_POINT('Ctrl Pts',(16.6211977614521,-18.7980430573374,-7.6982970139465));
#85506=CARTESIAN_POINT('Ctrl Pts',(16.6169831628437,-18.8752274520633,-7.6936766464845));
#85507=CARTESIAN_POINT('Ctrl Pts',(16.617000050606,-18.9524628884561,-7.6890562790225));
#85508=CARTESIAN_POINT('Ctrl Pts',(16.6203930087273,-18.9524685809736,-7.68905589348695));
#85509=CARTESIAN_POINT('Ctrl Pts',(16.6199117165189,-19.2000067410856,-7.67422393562464));
#85510=CARTESIAN_POINT('Ctrl Pts',(16.6606020197591,-19.4473941720768,-7.65939197776232));
#85511=CARTESIAN_POINT('Ctrl Pts',(16.7430902533864,-19.6789409674447,-7.64456001990001));
#85512=CARTESIAN_POINT('Origin',(18.734,-18.952,0.));
#85513=CARTESIAN_POINT('',(16.7454194485728,-19.6781104533646,-6.845005987876));
#85514=CARTESIAN_POINT('',(16.7454194581678,-19.6781104796424,-7.06814844662885));
#85515=CARTESIAN_POINT('',(16.7454194499637,-19.6781104571739,0.));
#85516=CARTESIAN_POINT('',(16.6170002518876,-18.9509672890084,-7.10922274860006));
#85517=CARTESIAN_POINT('Ctrl Pts',(16.7454194581678,-19.6781104796424,-7.06814844662885));
#85518=CARTESIAN_POINT('Ctrl Pts',(16.7207165638647,-19.6104572831724,-7.07229326072067));
#85519=CARTESIAN_POINT('Ctrl Pts',(16.6994767838628,-19.5415729101478,-7.07632982305453));
#85520=CARTESIAN_POINT('Ctrl Pts',(16.6386705851604,-19.3014695034662,-7.08999348029963));
#85521=CARTESIAN_POINT('Ctrl Pts',(16.6169146031621,-19.1265423838649,-7.0992095971379));
#85522=CARTESIAN_POINT('Ctrl Pts',(16.6170002518876,-18.9509672890084,-7.10922274860006));
#85523=CARTESIAN_POINT('Ctrl Pts',(16.617000253271,-18.9509644570508,-7.10922291010835));
#85524=CARTESIAN_POINT('Ctrl Pts',(16.6170133611986,-18.9241674230888,-7.11075116213054));
#85525=CARTESIAN_POINT('Ctrl Pts',(16.6175352641052,-18.8973740236385,-7.11229811087022));
#85526=CARTESIAN_POINT('Ctrl Pts',(16.6191227647428,-18.8561184599557,-7.11471892900856));
#85527=CARTESIAN_POINT('Ctrl Pts',(16.6198286092063,-18.8416446884933,-7.11557561664734));
#85528=CARTESIAN_POINT('Ctrl Pts',(16.620960018787,-18.8224889256946,-7.11672055060971));
#85529=CARTESIAN_POINT('Ctrl Pts',(16.6212526901732,-18.8177990892457,-7.11700174460842));
#85530=CARTESIAN_POINT('Ctrl Pts',(16.6217938177868,-18.8095688228847,-7.11749682870153));
#85531=CARTESIAN_POINT('Ctrl Pts',(16.622035569275,-18.8060279501914,-7.11771035080805));
#85532=CARTESIAN_POINT('Ctrl Pts',(16.6225281743189,-18.7990703883075,-7.11813096599797));
#85533=CARTESIAN_POINT('Ctrl Pts',(16.6227784202911,-18.7956536599959,-7.11833802549928));
#85534=CARTESIAN_POINT('Ctrl Pts',(16.6233330675064,-18.7883250307724,-7.11878325544969));
#85535=CARTESIAN_POINT('Ctrl Pts',(16.6236400496722,-18.7844133807662,-7.11902156683151));
#85536=CARTESIAN_POINT('Ctrl Pts',(16.62447652773,-18.7741216540878,-7.11965029844778));
#85537=CARTESIAN_POINT('Ctrl Pts',(16.6250240886659,-18.7677431439984,-7.12004171197717));
#85538=CARTESIAN_POINT('Ctrl Pts',(16.6274167974474,-18.7412797610905,-7.12167258776839));
#85539=CARTESIAN_POINT('Ctrl Pts',(16.6295199350736,-18.7212200268298,-7.1229254821994));
#85540=CARTESIAN_POINT('Ctrl Pts',(16.632414264621,-18.6969616360284,-7.12445836054343));
#85541=CARTESIAN_POINT('Ctrl Pts',(16.6329320498058,-18.6927305680807,-7.12472637581752));
#85542=CARTESIAN_POINT('Ctrl Pts',(16.6366907780554,-18.662767065183,-7.12662891591402));
#85543=CARTESIAN_POINT('Ctrl Pts',(16.6403914554856,-18.6370955500176,-7.12828251233134));
#85544=CARTESIAN_POINT('Ctrl Pts',(16.6729288516913,-18.437433946874,-7.141296005818));
#85545=CARTESIAN_POINT('Ctrl Pts',(16.722934133997,-18.2675918236132,-7.15319938306154));
#85546=CARTESIAN_POINT('Ctrl Pts',(16.8171419203852,-18.0515199209895,-7.16840078661708));
#85547=CARTESIAN_POINT('Ctrl Pts',(16.8431322770721,-17.9981501512624,-7.17216862668756));
#85548=CARTESIAN_POINT('Ctrl Pts',(16.8885290151137,-17.9141005654831,-7.17811565638349));
#85549=CARTESIAN_POINT('Ctrl Pts',(16.9065396945572,-17.882707019612,-7.18034034020732));
#85550=CARTESIAN_POINT('Ctrl Pts',(16.931074012134,-17.8423746993651,-7.18320477377927));
#85551=CARTESIAN_POINT('Ctrl Pts',(16.9368742870969,-17.8330050917248,-7.18387067969934));
#85552=CARTESIAN_POINT('Ctrl Pts',(16.9464487817368,-17.8178051899742,-7.18495183978114));
#85553=CARTESIAN_POINT('Ctrl Pts',(16.9501789443334,-17.8119475151765,-7.18536871101327));
#85554=CARTESIAN_POINT('Ctrl Pts',(16.9574233689125,-17.8006938120197,-7.18617006425167));
#85555=CARTESIAN_POINT('Ctrl Pts',(16.9609335551142,-17.7952952632404,-7.18655469184895));
#85556=CARTESIAN_POINT('Ctrl Pts',(16.9690493356662,-17.7829372145805,-7.18743568328244));
#85557=CARTESIAN_POINT('Ctrl Pts',(16.9736715784317,-17.7759887351528,-7.18793141684298));
#85558=CARTESIAN_POINT('Ctrl Pts',(16.9861098378325,-17.7575283223654,-7.18924961557565));
#85559=CARTESIAN_POINT('Ctrl Pts',(16.9939985475541,-17.7460656871364,-7.1900693325874));
#85560=CARTESIAN_POINT('Ctrl Pts',(17.0581390682346,-17.6548065895051,-7.19660723570976));
#85561=CARTESIAN_POINT('Ctrl Pts',(17.1197399411334,-17.5789054841399,-7.20210985633664));
#85562=CARTESIAN_POINT('Ctrl Pts',(17.2799634000678,-17.4072401993666,-7.21506336376851));
#85563=CARTESIAN_POINT('Ctrl Pts',(17.3830793570561,-17.3162994579983,-7.22236047349061));
#85564=CARTESIAN_POINT('Ctrl Pts',(17.535963248145,-17.2058489698827,-7.23281030874296));
#85565=CARTESIAN_POINT('Ctrl Pts',(17.5787448784982,-17.1772548435322,-7.2357023421666));
#85566=CARTESIAN_POINT('Ctrl Pts',(17.6378691584124,-17.140781808804,-7.23971580381614));
#85567=CARTESIAN_POINT('Ctrl Pts',(17.6533358911243,-17.131511275045,-7.24076721868491));
#85568=CARTESIAN_POINT('Ctrl Pts',(17.6763955712468,-17.1180870459139,-7.2423398754025));
#85569=CARTESIAN_POINT('Ctrl Pts',(17.6838989937448,-17.1137802846113,-7.24285238914577));
#85570=CARTESIAN_POINT('Ctrl Pts',(17.6975309911582,-17.1060665887894,-7.24378531425949));
#85571=CARTESIAN_POINT('Ctrl Pts',(17.7036505379642,-17.1026438558614,-7.24420476686297));
#85572=CARTESIAN_POINT('Ctrl Pts',(17.7133176302825,-17.0972998150672,-7.24486858516731));
#85573=CARTESIAN_POINT('Ctrl Pts',(17.7168539213188,-17.0953581040382,-7.24511166736501));
#85574=CARTESIAN_POINT('Ctrl Pts',(17.7204047838171,-17.0934215814666,-7.24535602607436));
#85575=CARTESIAN_POINT('Ctrl Pts',(17.7204138606574,-17.0934166313454,-7.24535665071454));
#85576=CARTESIAN_POINT('Ctrl Pts',(17.7204320698581,-17.0934067009977,-7.24535790381921));
#85577=CARTESIAN_POINT('Ctrl Pts',(17.7204412018053,-17.0934017209977,-7.2453585322553));
#85578=CARTESIAN_POINT('Ctrl Pts',(17.7204595211243,-17.0933917309476,-7.24535979294531));
#85579=CARTESIAN_POINT('Ctrl Pts',(17.7204687089969,-17.0933867206256,-7.2453604252337));
#85580=CARTESIAN_POINT('Ctrl Pts',(17.7204871404368,-17.0933766697873,-7.24536169364699));
#85581=CARTESIAN_POINT('Ctrl Pts',(17.7204963842381,-17.0933716291446,-7.24536232978799));
#85582=CARTESIAN_POINT('Ctrl Pts',(17.7205149285648,-17.0933615171072,-7.24536360597739));
#85583=CARTESIAN_POINT('Ctrl Pts',(17.7205242285134,-17.0933564460279,-7.24536424598611));
#85584=CARTESIAN_POINT('Ctrl Pts',(17.7205428852673,-17.0933462730484,-7.24536552992014));
#85585=CARTESIAN_POINT('Ctrl Pts',(17.7205522423073,-17.0933411710211,-7.24536617386162));
#85586=CARTESIAN_POINT('Ctrl Pts',(17.7205710139306,-17.0933309357744,-7.24536746570849));
#85587=CARTESIAN_POINT('Ctrl Pts',(17.720580427922,-17.0933258028788,-7.24536811357317));
#85588=CARTESIAN_POINT('Ctrl Pts',(17.7205993135353,-17.0933155058512,-7.2453694132725));
#85589=CARTESIAN_POINT('Ctrl Pts',(17.7206087854619,-17.0933103415542,-7.24537006512815));
#85590=CARTESIAN_POINT('Ctrl Pts',(17.7206277871157,-17.0932999816346,-7.2453713728212));
#85591=CARTESIAN_POINT('Ctrl Pts',(17.7206373170627,-17.0932947858932,-7.24537202867376));
#85592=CARTESIAN_POINT('Ctrl Pts',(17.7206564352576,-17.0932843628154,-7.24537334439513));
#85593=CARTESIAN_POINT('Ctrl Pts',(17.7206660236408,-17.0932791354065,-7.24537400427328));
#85594=CARTESIAN_POINT('Ctrl Pts',(17.7206852592978,-17.0932686486756,-7.2453753280865));
#85595=CARTESIAN_POINT('Ctrl Pts',(17.7206949064925,-17.0932633893979,-7.24537599201615));
#85596=CARTESIAN_POINT('Ctrl Pts',(17.7207142599682,-17.0932528388266,-7.24537732394591));
#85597=CARTESIAN_POINT('Ctrl Pts',(17.7207239666169,-17.0932475473335,-7.24537799197136));
#85598=CARTESIAN_POINT('Ctrl Pts',(17.7207434019682,-17.0932369525225,-7.24537932954415));
#85599=CARTESIAN_POINT('Ctrl Pts',(17.7207531870614,-17.0932316184647,-7.24538000297263));
#85600=CARTESIAN_POINT('Ctrl Pts',(17.7207727992919,-17.0932209276323,-7.24538135272692));
#85601=CARTESIAN_POINT('Ctrl Pts',(17.720782625299,-17.093215571474,-7.24538202897517));
#85602=CARTESIAN_POINT('Ctrl Pts',(17.7208023394488,-17.0932048254899,-7.24538338575223));
#85603=CARTESIAN_POINT('Ctrl Pts',(17.7208122258835,-17.0931994365966,-7.2453840661635));
#85604=CARTESIAN_POINT('Ctrl Pts',(17.7208320614158,-17.0931886248587,-7.245385431303));
#85605=CARTESIAN_POINT('Ctrl Pts',(17.7208420089104,-17.0931832028893,-7.2453861159209));
#85606=CARTESIAN_POINT('Ctrl Pts',(17.7208619996744,-17.0931723069557,-7.2453874917526));
#85607=CARTESIAN_POINT('Ctrl Pts',(17.7208719923007,-17.0931668605965,-7.24538817948079));
#85608=CARTESIAN_POINT('Ctrl Pts',(17.7238842193324,-17.0915251142421,-7.24559549240892));
#85609=CARTESIAN_POINT('Ctrl Pts',(17.7268903493805,-17.0898961248331,-7.24580258652638));
#85610=CARTESIAN_POINT('Ctrl Pts',(17.7339397814265,-17.0860981773077,-7.24628868545938));
#85611=CARTESIAN_POINT('Ctrl Pts',(17.73798618483,-17.0839350836294,-7.24656805799393));
#85612=CARTESIAN_POINT('Ctrl Pts',(17.7504630090659,-17.0773173859405,-7.2474304842157));
#85613=CARTESIAN_POINT('Ctrl Pts',(17.7589163827721,-17.0729066421298,-7.24801619947914));
#85614=CARTESIAN_POINT('Ctrl Pts',(17.8726190897224,-17.0145534441301,-7.25591016519681));
#85615=CARTESIAN_POINT('Ctrl Pts',(17.9821673160887,-16.9694719843812,-7.26368497769928));
#85616=CARTESIAN_POINT('Ctrl Pts',(18.199216489691,-16.9007391822163,-7.27872419300949));
#85617=CARTESIAN_POINT('Ctrl Pts',(18.305955198866,-16.8758387687581,-7.28596054281728));
#85618=CARTESIAN_POINT('Ctrl Pts',(18.4890359883618,-16.8478562113822,-7.29786573935853));
#85619=CARTESIAN_POINT('Ctrl Pts',(18.5644921174166,-16.8404371346402,-7.30263387129201));
#85620=CARTESIAN_POINT('Ctrl Pts',(18.6590783958438,-16.8362417025176,-7.3084345722606));
#85621=CARTESIAN_POINT('Ctrl Pts',(18.6779762187534,-16.8356569766535,-7.30958494753696));
#85622=CARTESIAN_POINT('Ctrl Pts',(18.7054508277715,-16.8351751538426,-7.31124541240657));
#85623=CARTESIAN_POINT('Ctrl Pts',(18.7140227529653,-16.8350769032575,-7.31176177211313));
#85624=CARTESIAN_POINT('Ctrl Pts',(18.7290470400866,-16.8349959621119,-7.31266390696164));
#85625=CARTESIAN_POINT('Ctrl Pts',(18.7354991217446,-16.8349906985774,-7.31305038402281));
#85626=CARTESIAN_POINT('Ctrl Pts',(18.7480234389187,-16.8350377386504,-7.31379879919102));
#85627=CARTESIAN_POINT('Ctrl Pts',(18.7540956170281,-16.8350866715485,-7.31416083903772));
#85628=CARTESIAN_POINT('Ctrl Pts',(18.7686043123388,-16.8352660225221,-7.31502398017245));
#85629=CARTESIAN_POINT('Ctrl Pts',(18.777040467128,-16.8354207524491,-7.31552431696063));
#85630=CARTESIAN_POINT('Ctrl Pts',(18.8074392554409,-16.8361601277919,-7.31732185571079));
#85631=CARTESIAN_POINT('Ctrl Pts',(18.8293938734943,-16.8370362293236,-7.31860994896036));
#85632=CARTESIAN_POINT('Ctrl Pts',(19.0379766845316,-16.848614410365,-7.33076152277251));
#85633=CARTESIAN_POINT('Ctrl Pts',(19.2224218394706,-16.8836473321735,-7.34075359847646));
#85634=CARTESIAN_POINT('Ctrl Pts',(19.4751177952318,-16.96738027662,-7.35526996369034));
#85635=CARTESIAN_POINT('Ctrl Pts',(19.548889158123,-16.9965141948136,-7.35963130817193));
#85636=CARTESIAN_POINT('Ctrl Pts',(19.6533465863166,-17.0447056169168,-7.36621325344225));
#85637=CARTESIAN_POINT('Ctrl Pts',(19.6854582623626,-17.0605199334064,-7.36829547362044));
#85638=CARTESIAN_POINT('Ctrl Pts',(19.7237508746885,-17.080600060355,-7.3708687007561));
#85639=CARTESIAN_POINT('Ctrl Pts',(19.7303318437116,-17.0840954570668,-7.37131421667079));
#85640=CARTESIAN_POINT('Ctrl Pts',(19.7405543034133,-17.0895943761088,-7.37201159214417));
#85641=CARTESIAN_POINT('Ctrl Pts',(19.744208654356,-17.0915740413541,-7.37226196105825));
#85642=CARTESIAN_POINT('Ctrl Pts',(19.7509877783966,-17.0952723472187,-7.37272845052502));
#85643=CARTESIAN_POINT('Ctrl Pts',(19.7541140468696,-17.0969881270511,-7.37294438864439));
#85644=CARTESIAN_POINT('Ctrl Pts',(19.7611884180731,-17.1008940230815,-7.37343486583595));
#85645=CARTESIAN_POINT('Ctrl Pts',(19.7651338393522,-17.1030888640941,-7.37370970392245));
#85646=CARTESIAN_POINT('Ctrl Pts',(19.7753093798818,-17.1087922255504,-7.37442182568733));
#85647=CARTESIAN_POINT('Ctrl Pts',(19.7815287405006,-17.1123196856743,-7.37486028233949));
#85648=CARTESIAN_POINT('Ctrl Pts',(19.8197545465749,-17.1342570572481,-7.37757438090023));
#85649=CARTESIAN_POINT('Ctrl Pts',(19.8512906116546,-17.1534690301272,-7.37989686263477));
#85650=CARTESIAN_POINT('Ctrl Pts',(20.0255444227163,-17.2659773465048,-7.39313679436249));
#85651=CARTESIAN_POINT('Ctrl Pts',(20.1570850951643,-17.3754241632414,-7.40464131185876));
#85652=CARTESIAN_POINT('Ctrl Pts',(20.3393638462973,-17.5686887408063,-7.42190384273487));
#85653=CARTESIAN_POINT('Ctrl Pts',(20.3999164767335,-17.6422406198714,-7.42794872778959));
#85654=CARTESIAN_POINT('Ctrl Pts',(20.4677576804373,-17.7369980560549,-7.43510701715657));
#85655=CARTESIAN_POINT('Ctrl Pts',(20.479930989718,-17.7545567028381,-7.43640920745788));
#85656=CARTESIAN_POINT('Ctrl Pts',(20.4968549085228,-17.7797744825177,-7.43824590489082));
#85657=CARTESIAN_POINT('Ctrl Pts',(20.5018253344634,-17.7872838615844,-7.43878869632849));
#85658=CARTESIAN_POINT('Ctrl Pts',(20.5103146616573,-17.8002891834805,-7.43972170567695));
#85659=CARTESIAN_POINT('Ctrl Pts',(20.5138563151837,-17.8057700575856,-7.44011277287772));
#85660=CARTESIAN_POINT('Ctrl Pts',(20.520587165513,-17.8162927801484,-7.44085954613924));
#85661=CARTESIAN_POINT('Ctrl Pts',(20.5237804979782,-17.8213318968956,-7.441215403657));
#85662=CARTESIAN_POINT('Ctrl Pts',(20.5320248987022,-17.8344641066001,-7.44213827486938));
#85663=CARTESIAN_POINT('Ctrl Pts',(20.5370426746313,-17.8425780210501,-7.4427040549919));
#85664=CARTESIAN_POINT('Ctrl Pts',(20.5539458131906,-17.8703285704087,-7.44462431866771));
#85665=CARTESIAN_POINT('Ctrl Pts',(20.565566857233,-17.8901248883897,-7.4459691489453));
#85666=CARTESIAN_POINT('Ctrl Pts',(20.6634795157496,-18.0633093628527,-7.45753007006511));
#85667=CARTESIAN_POINT('Ctrl Pts',(20.7306536824789,-18.2267117827958,-7.46699016710072));
#85668=CARTESIAN_POINT('Ctrl Pts',(20.7995675841096,-18.4801663971577,-7.48128271780431));
#85669=CARTESIAN_POINT('Ctrl Pts',(20.8171447467062,-18.565086594589,-7.48602724678504));
#85670=CARTESIAN_POINT('Ctrl Pts',(20.8348366408193,-18.6881854330896,-7.49312839260848));
#85671=CARTESIAN_POINT('Ctrl Pts',(20.839204550445,-18.7256681167404,-7.49532030000414));
#85672=CARTESIAN_POINT('Ctrl Pts',(20.8432429871891,-18.770781146182,-7.49801516787105));
#85673=CARTESIAN_POINT('Ctrl Pts',(20.8438772085154,-18.7783209481372,-7.49846746253409));
#85674=CARTESIAN_POINT('Ctrl Pts',(20.8447991098677,-18.790032102848,-7.49917315517864));
#85675=CARTESIAN_POINT('Ctrl Pts',(20.8451148812046,-18.7942012687356,-7.49942500438653));
#85676=CARTESIAN_POINT('Ctrl Pts',(20.8456769241264,-18.801925787125,-7.49989282246133));
#85677=CARTESIAN_POINT('Ctrl Pts',(20.8459265695905,-18.8054808362956,-7.50010859985754));
#85678=CARTESIAN_POINT('Ctrl Pts',(20.8464698839516,-18.8135078558083,-7.50059687333769));
#85679=CARTESIAN_POINT('Ctrl Pts',(20.8467583282351,-18.8179801125796,-7.50086965698074));
#85680=CARTESIAN_POINT('Ctrl Pts',(20.847565721075,-18.8311494646103,-7.50167503304515));
#85681=CARTESIAN_POINT('Ctrl Pts',(20.8480451753326,-18.8398487634193,-7.50220975779561));
#85682=CARTESIAN_POINT('Ctrl Pts',(20.8510717496147,-18.9017109229873,-7.50603039148208));
#85683=CARTESIAN_POINT('Ctrl Pts',(20.8516666585363,-18.9549457950084,-7.50941293015124));
#85684=CARTESIAN_POINT('Ctrl Pts',(20.8497711832953,-19.0263960297577,-7.51403194162836));
#85685=CARTESIAN_POINT('Ctrl Pts',(20.849050744181,-19.0446433585941,-7.51521854577946));
#85686=CARTESIAN_POINT('Ctrl Pts',(20.8455799974383,-19.1108191534427,-7.5195424888418));
#85687=CARTESIAN_POINT('Ctrl Pts',(20.8414357445182,-19.1586590493085,-7.52270729218872));
#85688=CARTESIAN_POINT('Ctrl Pts',(20.822529538245,-19.3149004441581,-7.53310346283865));
#85689=CARTESIAN_POINT('Ctrl Pts',(20.8009934882782,-19.4223123959892,-7.54033585418034));
#85690=CARTESIAN_POINT('Ctrl Pts',(20.7562714471666,-19.580603704721,-7.55090864596328));
#85691=CARTESIAN_POINT('Ctrl Pts',(20.7392270189506,-19.6330211794603,-7.55439742641563));
#85692=CARTESIAN_POINT('Ctrl Pts',(20.7082836935235,-19.7168983166133,-7.55995449481805));
#85693=CARTESIAN_POINT('Ctrl Pts',(20.6956309787732,-19.7487870836441,-7.56206121286768));
#85694=CARTESIAN_POINT('Ctrl Pts',(20.6779792150162,-19.7903022293691,-7.56479758075175));
#85695=CARTESIAN_POINT('Ctrl Pts',(20.6736739501927,-19.8002162400644,-7.56545056847658));
#85696=CARTESIAN_POINT('Ctrl Pts',(20.6664968964457,-19.8164028730471,-7.56651604785952));
#85697=CARTESIAN_POINT('Ctrl Pts',(20.6636700781835,-19.8226951089903,-7.56693006884819));
#85698=CARTESIAN_POINT('Ctrl Pts',(20.6581377968209,-19.8348501733766,-7.56772958179424));
#85699=CARTESIAN_POINT('Ctrl Pts',(20.6554361697854,-19.840714654235,-7.56811520006939));
#85700=CARTESIAN_POINT('Ctrl Pts',(20.6491350499264,-19.8542295849077,-7.56900363049126));
#85701=CARTESIAN_POINT('Ctrl Pts',(20.6455164563949,-19.8618710476955,-7.56950577652471));
#85702=CARTESIAN_POINT('Ctrl Pts',(20.6356588493757,-19.882369191595,-7.57085242448115));
#85703=CARTESIAN_POINT('Ctrl Pts',(20.6293352079079,-19.895184858156,-7.57169398473442));
#85704=CARTESIAN_POINT('Ctrl Pts',(20.5701076035913,-20.0122156999669,-7.57937803238027));
#85705=CARTESIAN_POINT('Ctrl Pts',(20.508785386332,-20.1119528273776,-7.58590361758807));
#85706=CARTESIAN_POINT('Ctrl Pts',(20.3430318087841,-20.3373670978567,-7.60122072336177));
#85707=CARTESIAN_POINT('Ctrl Pts',(20.2317156437972,-20.4570120549477,-7.6098287101515));
#85708=CARTESIAN_POINT('Ctrl Pts',(20.0832086240643,-20.5836770448465,-7.62103837067635));
#85709=CARTESIAN_POINT('Ctrl Pts',(20.0581389034589,-20.6040864980786,-7.62292397217365));
#85710=CARTESIAN_POINT('Ctrl Pts',(20.026905799962,-20.6283459733375,-7.62527875170373));
#85711=CARTESIAN_POINT('Ctrl Pts',(20.0211756452397,-20.6327498578838,-7.62571099476218));
#85712=CARTESIAN_POINT('Ctrl Pts',(20.0121540464092,-20.6396101743367,-7.62639207054822));
#85713=CARTESIAN_POINT('Ctrl Pts',(20.0088777497708,-20.6420865626817,-7.62663952362488));
#85714=CARTESIAN_POINT('Ctrl Pts',(20.0027381899975,-20.6466991375734,-7.62710348726891));
#85715=CARTESIAN_POINT('Ctrl Pts',(19.9998767187544,-20.6488376156566,-7.62731983349712));
#85716=CARTESIAN_POINT('Ctrl Pts',(19.9933296662705,-20.6537046806974,-7.62781506717365));
#85717=CARTESIAN_POINT('Ctrl Pts',(19.9896406359132,-20.6564285321438,-7.62809427792971));
#85718=CARTESIAN_POINT('Ctrl Pts',(19.9782646328368,-20.664771200313,-7.62895571946072));
#85719=CARTESIAN_POINT('Ctrl Pts',(19.9705487028104,-20.6703500688002,-7.62954060318709));
#85720=CARTESIAN_POINT('Ctrl Pts',(19.8652733990393,-20.7453913035297,-7.63752583935986));
#85721=CARTESIAN_POINT('Ctrl Pts',(19.7620392319504,-20.8064973880513,-7.64540431265029));
#85722=CARTESIAN_POINT('Ctrl Pts',(19.5561164994488,-20.9058876651664,-7.66050997952928));
#85723=CARTESIAN_POINT('Ctrl Pts',(19.4545093650631,-20.9455953148074,-7.66770930842107));
#85724=CARTESIAN_POINT('Ctrl Pts',(19.2785781956098,-20.9991303388827,-7.67952435461965));
#85725=CARTESIAN_POINT('Ctrl Pts',(19.205750333317,-21.0171299713888,-7.68424034705386));
#85726=CARTESIAN_POINT('Ctrl Pts',(19.1136512399724,-21.0347643378857,-7.68998480594451));
#85727=CARTESIAN_POINT('Ctrl Pts',(19.0951422709268,-21.0380533663137,-7.69112852502209));
#85728=CARTESIAN_POINT('Ctrl Pts',(19.0681517051492,-21.0424795581679,-7.69278120577576));
#85729=CARTESIAN_POINT('Ctrl Pts',(19.059703537322,-21.0438124567707,-7.69329635533019));
#85730=CARTESIAN_POINT('Ctrl Pts',(19.0448713257135,-21.0460605548708,-7.69419709358531));
#85731=CARTESIAN_POINT('Ctrl Pts',(19.0384907888664,-21.0469978399845,-7.69458337756545));
#85732=CARTESIAN_POINT('Ctrl Pts',(19.0260884675414,-21.0487618535583,-7.69533193958978));
#85733=CARTESIAN_POINT('Ctrl Pts',(19.0200672159361,-21.0495918317346,-7.69569431692425));
#85734=CARTESIAN_POINT('Ctrl Pts',(19.0056573295866,-21.0515149100075,-7.69655909101826));
#85735=CARTESIAN_POINT('Ctrl Pts',(18.9972655118182,-21.0525836892411,-7.69706071659597));
#85736=CARTESIAN_POINT('Ctrl Pts',(18.9669181698148,-21.0562639998756,-7.69886774890163));
#85737=CARTESIAN_POINT('Ctrl Pts',(18.9449279887498,-21.0585818979752,-7.70016391874448));
#85738=CARTESIAN_POINT('Ctrl Pts',(18.7380773542932,-21.0771135936689,-7.71224252135256));
#85739=CARTESIAN_POINT('Ctrl Pts',(18.5518804069917,-21.0693008479196,-7.72216856688949));
#85740=CARTESIAN_POINT('Ctrl Pts',(18.2612635610973,-21.0184434176323,-7.73825201626216));
#85741=CARTESIAN_POINT('Ctrl Pts',(18.155091895123,-20.9912467067075,-7.74428538351675));
#85742=CARTESIAN_POINT('Ctrl Pts',(18.0403466907054,-20.9521683076997,-7.75143993975321));
#85743=CARTESIAN_POINT('Ctrl Pts',(18.0292116778076,-20.9482719201642,-7.75214109640204));
#85744=CARTESIAN_POINT('Ctrl Pts',(18.0134012884487,-20.942590749691,-7.75314724322877));
#85745=CARTESIAN_POINT('Ctrl Pts',(18.0086985461336,-20.940882056758,-7.75344785950515));
#85746=CARTESIAN_POINT('Ctrl Pts',(18.0005943822121,-20.9379049268266,-7.75396829664887));
#85747=CARTESIAN_POINT('Ctrl Pts',(17.9971900495196,-20.9366443699878,-7.75418764843126));
#85748=CARTESIAN_POINT('Ctrl Pts',(17.9905874773202,-20.9341802386042,-7.7546145190964));
#85749=CARTESIAN_POINT('Ctrl Pts',(17.9873889037563,-20.9329776747283,-7.75482197166372));
#85750=CARTESIAN_POINT('Ctrl Pts',(17.9787493745823,-20.929705584748,-7.755384065364));
#85751=CARTESIAN_POINT('Ctrl Pts',(17.9733140678972,-20.9276213701007,-7.75573957307488));
#85752=CARTESIAN_POINT('Ctrl Pts',(17.9530708093983,-20.9197629981159,-7.75707047437662));
#85753=CARTESIAN_POINT('Ctrl Pts',(17.9383198625403,-20.9138447190879,-7.75805398748051));
#85754=CARTESIAN_POINT('Ctrl Pts',(17.8094424093461,-20.8604448132691,-7.76675887775666));
#85755=CARTESIAN_POINT('Ctrl Pts',(17.6996216082782,-20.8032222864274,-7.77493827884515));
#85756=CARTESIAN_POINT('Ctrl Pts',(17.4545040878102,-20.646851667991,-7.79415151237519));
#85757=CARTESIAN_POINT('Ctrl Pts',(17.3246942560686,-20.5405559789002,-7.80506941645519));
#85758=CARTESIAN_POINT('Ctrl Pts',(17.1939623449152,-20.4047307047863,-7.81664815580069));
#85759=CARTESIAN_POINT('Ctrl Pts',(17.1794268214328,-20.3891655312427,-7.81794608731221));
#85760=CARTESIAN_POINT('Ctrl Pts',(17.1590898587272,-20.3667183215896,-7.81977787410395));
#85761=CARTESIAN_POINT('Ctrl Pts',(17.1530939780275,-20.3600149275195,-7.82031995357325));
#85762=CARTESIAN_POINT('Ctrl Pts',(17.1428230022233,-20.3483836565338,-7.82125212340098));
#85763=CARTESIAN_POINT('Ctrl Pts',(17.1385276683435,-20.3434738929946,-7.82164305901465));
#85764=CARTESIAN_POINT('Ctrl Pts',(17.1303462116784,-20.334034422648,-7.82238984245075));
#85765=CARTESIAN_POINT('Ctrl Pts',(17.1264564218029,-20.329507990359,-7.82274584047264));
#85766=CARTESIAN_POINT('Ctrl Pts',(17.116390082127,-20.3176933838864,-7.82366964147331));
#85767=CARTESIAN_POINT('Ctrl Pts',(17.1102435877225,-20.3103796904132,-7.82423620585244));
#85768=CARTESIAN_POINT('Ctrl Pts',(17.0894465473258,-20.285290491069,-7.82616203298827));
#85769=CARTESIAN_POINT('Ctrl Pts',(17.0750363784865,-20.2673172073819,-7.82751156515189));
#85770=CARTESIAN_POINT('Ctrl Pts',(16.9537660341881,-20.1108968052215,-7.83901211840196));
#85771=CARTESIAN_POINT('Ctrl Pts',(16.8641495643365,-19.959938913254,-7.84841817815766));
#85772=CARTESIAN_POINT('Ctrl Pts',(16.7766289145641,-19.7596475759913,-7.86031011867401));
#85773=CARTESIAN_POINT('Ctrl Pts',(16.7603899223379,-19.7191097138761,-7.86269367145722));
#85774=CARTESIAN_POINT('Ctrl Pts',(16.7454194590822,-19.6781104821466,-7.86510586795993));
#85775=CARTESIAN_POINT('',(16.6156461116265,-18.9537405764281,-6.88905704663589));
#85776=CARTESIAN_POINT('Ctrl Pts',(16.7430902533864,-19.6789409674447,-7.64456001990001));
#85777=CARTESIAN_POINT('Ctrl Pts',(16.7690655542301,-19.7518543685999,-7.63988948022869));
#85778=CARTESIAN_POINT('Ctrl Pts',(17.0725682270039,-20.4707351681624,-7.5928270049969));
#85779=CARTESIAN_POINT('Ctrl Pts',(18.4531255376191,-21.4394563861295,-7.50337259420462));
#85780=CARTESIAN_POINT('Ctrl Pts',(20.673525152946,-20.5345839369853,-7.3761967875232));
#85781=CARTESIAN_POINT('Ctrl Pts',(21.1145308209525,-18.1777889518937,-7.24902098084176));
#85782=CARTESIAN_POINT('Ctrl Pts',(19.371547213141,-16.5312845504829,-7.12184517416032));
#85783=CARTESIAN_POINT('Ctrl Pts',(17.1752234457631,-17.0731746333353,-7.00185719609169));
#85784=CARTESIAN_POINT('Ctrl Pts',(16.6208560643663,-18.3695361560074,-6.92426115358356));
#85785=CARTESIAN_POINT('Ctrl Pts',(16.6156461116265,-18.9537405764281,-6.88905704663589));
#85786=CARTESIAN_POINT('Ctrl Pts',(16.6170007608245,-18.9537948065389,-6.88983560106466));
#85787=CARTESIAN_POINT('Ctrl Pts',(16.6170691195685,-19.0344248943613,-6.88542677740563));
#85788=CARTESIAN_POINT('Ctrl Pts',(16.6217438746711,-19.1149800361354,-6.8809632257301));
#85789=CARTESIAN_POINT('Ctrl Pts',(16.6337248070316,-19.2186387330682,-6.8749301875487));
#85790=CARTESIAN_POINT('Ctrl Pts',(16.6368453937014,-19.2421629775274,-6.87354145267081));
#85791=CARTESIAN_POINT('Ctrl Pts',(16.6412432763108,-19.2715211984353,-6.87177821045316));
#85792=CARTESIAN_POINT('Ctrl Pts',(16.6421508389439,-19.2774098743235,-6.8714230179003));
#85793=CARTESIAN_POINT('Ctrl Pts',(16.6437157810073,-19.2872867753239,-6.87082459126562));
#85794=CARTESIAN_POINT('Ctrl Pts',(16.6443597521227,-19.2912771311432,-6.87058208819888));
#85795=CARTESIAN_POINT('Ctrl Pts',(16.6455594684996,-19.2985781525279,-6.87013700514065));
#85796=CARTESIAN_POINT('Ctrl Pts',(16.6461116701162,-19.3018893982353,-6.86993462430001));
#85797=CARTESIAN_POINT('Ctrl Pts',(16.6472681666741,-19.3087240324362,-6.86951579339881));
#85798=CARTESIAN_POINT('Ctrl Pts',(16.6478735059419,-19.3122471785425,-6.86929928258382));
#85799=CARTESIAN_POINT('Ctrl Pts',(16.6492800583166,-19.3203110435557,-6.86880233975892));
#85800=CARTESIAN_POINT('Ctrl Pts',(16.6500871820472,-19.3248506756071,-6.86852157583359));
#85801=CARTESIAN_POINT('Ctrl Pts',(16.6526294580089,-19.3388834421341,-6.86765065397933));
#85802=CARTESIAN_POINT('Ctrl Pts',(16.6544146688601,-19.3483672202379,-6.86705775947629));
#85803=CARTESIAN_POINT('Ctrl Pts',(16.6734315752866,-19.4457264490839,-6.86092926727658));
#85804=CARTESIAN_POINT('Ctrl Pts',(16.6961558852748,-19.532427133864,-6.85512342797589));
#85805=CARTESIAN_POINT('Ctrl Pts',(16.7310304511555,-19.6377557645575,-6.8478320303573));
#85806=CARTESIAN_POINT('Ctrl Pts',(16.7380722943999,-19.6579889858539,-6.8464199563341));
#85807=CARTESIAN_POINT('Ctrl Pts',(16.7454194485728,-19.6781104533646,-6.84500598787601));
#85808=CARTESIAN_POINT('Origin',(18.734,-18.952,0.));
#85809=CARTESIAN_POINT('',(16.745419449956,-19.6781104571528,-6.04247203196383));
#85810=CARTESIAN_POINT('',(16.7454195726558,-19.6781107931876,-6.26710635146282));
#85811=CARTESIAN_POINT('',(16.7454194499637,-19.6781104571739,0.));
#85812=CARTESIAN_POINT('Ctrl Pts',(16.7454195726558,-19.6781107931876,-6.26710635146282));
#85813=CARTESIAN_POINT('Ctrl Pts',(16.7157171117681,-19.5967654490344,-6.27277684093396));
#85814=CARTESIAN_POINT('Ctrl Pts',(16.691004302357,-19.5135927381583,-6.27836338234672));
#85815=CARTESIAN_POINT('Ctrl Pts',(16.6614520768127,-19.3858238017327,-6.28658112014348));
#85816=CARTESIAN_POINT('Ctrl Pts',(16.6528139473508,-19.3422858750625,-6.28932035095603));
#85817=CARTESIAN_POINT('Ctrl Pts',(16.6436144425346,-19.2868388967681,-6.29273464287481));
#85818=CARTESIAN_POINT('Ctrl Pts',(16.6417764795419,-19.2751557132193,-6.29344995119706));
#85819=CARTESIAN_POINT('Ctrl Pts',(16.6389885133478,-19.256411908666,-6.29459111071411));
#85820=CARTESIAN_POINT('Ctrl Pts',(16.6379760965532,-19.2493609548218,-6.29501893121541));
#85821=CARTESIAN_POINT('Ctrl Pts',(16.6361227659771,-19.235973530818,-6.29582850592141));
#85822=CARTESIAN_POINT('Ctrl Pts',(16.6352749264707,-19.2296381140277,-6.29621047502385));
#85823=CARTESIAN_POINT('Ctrl Pts',(16.6334140696412,-19.2152372035021,-6.29707615108004));
#85824=CARTESIAN_POINT('Ctrl Pts',(16.6324187832403,-19.2071694893753,-6.29755929335929));
#85825=CARTESIAN_POINT('Ctrl Pts',(16.6299653953218,-19.1862937224656,-6.29880484378213));
#85826=CARTESIAN_POINT('Ctrl Pts',(16.6285777511622,-19.173477608704,-6.29956503076248));
#85827=CARTESIAN_POINT('Ctrl Pts',(16.6203967172938,-19.0908752883665,-6.30443700703756));
#85828=CARTESIAN_POINT('Ctrl Pts',(16.6169563815645,-19.0207966549477,-6.30844166709839));
#85829=CARTESIAN_POINT('Ctrl Pts',(16.6171212273236,-18.7582834317184,-6.3231406527529));
#85830=CARTESIAN_POINT('Ctrl Pts',(16.6434647838365,-18.5668343991246,-6.33317498122216));
#85831=CARTESIAN_POINT('Ctrl Pts',(16.7087052288393,-18.3336573108351,-6.34683370371062));
#85832=CARTESIAN_POINT('Ctrl Pts',(16.7238020870876,-18.2862146758212,-6.34969720243455));
#85833=CARTESIAN_POINT('Ctrl Pts',(16.743184512298,-18.2319974294047,-6.35311511291673));
#85834=CARTESIAN_POINT('Ctrl Pts',(16.7458544887832,-18.2246572818048,-6.35358098216849));
#85835=CARTESIAN_POINT('Ctrl Pts',(16.7501831753964,-18.2129590338692,-6.35432872963475));
#85836=CARTESIAN_POINT('Ctrl Pts',(16.7518158007495,-18.2085912682182,-6.35460909533752));
#85837=CARTESIAN_POINT('Ctrl Pts',(16.754731033288,-18.2008700189836,-6.35510687067238));
#85838=CARTESIAN_POINT('Ctrl Pts',(16.7560077573588,-18.1975143613936,-6.35532392675766));
#85839=CARTESIAN_POINT('Ctrl Pts',(16.7587298593755,-18.1904141665802,-6.35578474685558));
#85840=CARTESIAN_POINT('Ctrl Pts',(16.7601773291144,-18.1866705458515,-6.35602862985684));
#85841=CARTESIAN_POINT('Ctrl Pts',(16.7641078965034,-18.1765901591777,-6.35668774850972));
#85842=CARTESIAN_POINT('Ctrl Pts',(16.7666108958845,-18.1702612771773,-6.35710415327289));
#85843=CARTESIAN_POINT('Ctrl Pts',(16.7791207435806,-18.1390705163343,-6.35916871338343));
#85844=CARTESIAN_POINT('Ctrl Pts',(16.7895680732758,-18.1143893628866,-6.36084134111789));
#85845=CARTESIAN_POINT('Ctrl Pts',(16.8210382304209,-18.0438068432985,-6.36572420168939));
#85846=CARTESIAN_POINT('Ctrl Pts',(16.8432373491214,-17.998452172392,-6.36898504072832));
#85847=CARTESIAN_POINT('Ctrl Pts',(16.9295816986985,-17.8369373174763,-6.38094757349529));
#85848=CARTESIAN_POINT('Ctrl Pts',(17.0029893224962,-17.7260737688442,-6.38981577853393));
#85849=CARTESIAN_POINT('Ctrl Pts',(17.1511163108997,-17.5424515436706,-6.40514170336334));
#85850=CARTESIAN_POINT('Ctrl Pts',(17.2217357934411,-17.4669376859675,-6.41168264531775));
#85851=CARTESIAN_POINT('Ctrl Pts',(17.3079107814179,-17.3873416524933,-6.41884329591353));
#85852=CARTESIAN_POINT('Ctrl Pts',(17.3183213355733,-17.377916095698,-6.4196961042375));
#85853=CARTESIAN_POINT('Ctrl Pts',(17.3350950525198,-17.3630304533005,-6.42105099683033));
#85854=CARTESIAN_POINT('Ctrl Pts',(17.3413980605459,-17.3575034920675,-6.42155588183445));
#85855=CARTESIAN_POINT('Ctrl Pts',(17.3526049401324,-17.3477935828225,-6.42244618259143));
#85856=CARTESIAN_POINT('Ctrl Pts',(17.3574953665302,-17.3435953445102,-6.422832231047));
#85857=CARTESIAN_POINT('Ctrl Pts',(17.3676822004434,-17.3349308400779,-6.4236313332911));
#85858=CARTESIAN_POINT('Ctrl Pts',(17.3729815188126,-17.3304681030036,-6.42404423919218));
#85859=CARTESIAN_POINT('Ctrl Pts',(17.3867089413886,-17.319022476089,-6.42510671568596));
#85860=CARTESIAN_POINT('Ctrl Pts',(17.3951695289611,-17.3120787315126,-6.42575468847182));
#85861=CARTESIAN_POINT('Ctrl Pts',(17.4313068415752,-17.2828863101937,-6.42849389265831));
#85862=CARTESIAN_POINT('Ctrl Pts',(17.4594881367251,-17.2612694767678,-6.43055978551352));
#85863=CARTESIAN_POINT('Ctrl Pts',(17.5349316974395,-17.2063583422862,-6.43592259260299));
#85864=CARTESIAN_POINT('Ctrl Pts',(17.5830376397931,-17.1742722467271,-6.43917557627524));
#85865=CARTESIAN_POINT('Ctrl Pts',(17.7707935587747,-17.0598617589398,-6.45137509240044));
#85866=CARTESIAN_POINT('Ctrl Pts',(17.9184023092571,-16.9917069730889,-6.45992612549223));
#85867=CARTESIAN_POINT('Ctrl Pts',(18.0929231656286,-16.9342836115624,-6.47018705162299));
#85868=CARTESIAN_POINT('Ctrl Pts',(18.1136173423145,-16.927825047436,-6.47140679620249));
#85869=CARTESIAN_POINT('Ctrl Pts',(18.1746816658197,-16.9097914988215,-6.4750244682675));
#85870=CARTESIAN_POINT('Ctrl Pts',(18.21529888653,-16.8990993237991,-6.47745422207117));
#85871=CARTESIAN_POINT('Ctrl Pts',(18.2634492315649,-16.887944214515,-6.48039067514367));
#85872=CARTESIAN_POINT('Ctrl Pts',(18.2707031673798,-16.8863039060714,-6.48083454203317));
#85873=CARTESIAN_POINT('Ctrl Pts',(18.2824592564999,-16.8837105778642,-6.481556517014));
#85874=CARTESIAN_POINT('Ctrl Pts',(18.2869562101733,-16.8827339403016,-6.4818333072944));
#85875=CARTESIAN_POINT('Ctrl Pts',(18.2949512122112,-16.8810248831129,-6.4823265620341));
#85876=CARTESIAN_POINT('Ctrl Pts',(18.2984479674057,-16.8802866512211,-6.48254269046489));
#85877=CARTESIAN_POINT('Ctrl Pts',(18.3059568251153,-16.878721238935,-6.48300766352775));
#85878=CARTESIAN_POINT('Ctrl Pts',(18.3099694042507,-16.8778968603612,-6.4832566586424));
#85879=CARTESIAN_POINT('Ctrl Pts',(18.321020868464,-16.875659763212,-6.48394383287429));
#85880=CARTESIAN_POINT('Ctrl Pts',(18.3280645101896,-16.8742712119483,-6.48438335376392));
#85881=CARTESIAN_POINT('Ctrl Pts',(18.3661873357337,-16.8669571047216,-6.48677007694406));
#85882=CARTESIAN_POINT('Ctrl Pts',(18.3973875683389,-16.8616933590456,-6.48875161386752));
#85883=CARTESIAN_POINT('Ctrl Pts',(18.5904532894668,-16.8335557954143,-6.501138798924));
#85884=CARTESIAN_POINT('Ctrl Pts',(18.7543959575774,-16.8287959773175,-6.51214903693729));
#85885=CARTESIAN_POINT('Ctrl Pts',(19.033862890239,-16.8530783698959,-6.53047401592194));
#85886=CARTESIAN_POINT('Ctrl Pts',(19.1494470394382,-16.8728652348922,-6.53793076193387));
#85887=CARTESIAN_POINT('Ctrl Pts',(19.2766584581424,-16.9056825582303,-6.54595262162781));
#85888=CARTESIAN_POINT('Ctrl Pts',(19.2904615806804,-16.9093928915137,-6.54682078999123));
#85889=CARTESIAN_POINT('Ctrl Pts',(19.3123692531386,-16.9155203165439,-6.54819534458157));
#85890=CARTESIAN_POINT('Ctrl Pts',(19.3204985382494,-16.9178466227992,-6.5487046605073));
#85891=CARTESIAN_POINT('Ctrl Pts',(19.3348107017058,-16.9220351747256,-6.54960010301336));
#85892=CARTESIAN_POINT('Ctrl Pts',(19.3409993653486,-16.9238771084979,-6.54998688601738));
#85893=CARTESIAN_POINT('Ctrl Pts',(19.3537815728068,-16.9277452284498,-6.55078494255546));
#85894=CARTESIAN_POINT('Ctrl Pts',(19.36037384217,-16.9297753859397,-6.55119608086406));
#85895=CARTESIAN_POINT('Ctrl Pts',(19.3772687660389,-16.9350688942401,-6.55224867059282));
#85896=CARTESIAN_POINT('Ctrl Pts',(19.3875566481281,-16.9383790066186,-6.55288858140185));
#85897=CARTESIAN_POINT('Ctrl Pts',(19.4303800315285,-16.9525201443215,-6.5555482941823));
#85898=CARTESIAN_POINT('Ctrl Pts',(19.4626763810054,-16.9640624331487,-6.55754458891593));
#85899=CARTESIAN_POINT('Ctrl Pts',(19.5460741881547,-16.9961734429723,-6.5626860350182));
#85900=CARTESIAN_POINT('Ctrl Pts',(19.5966794607789,-17.0179610136745,-6.56579185022321));
#85901=CARTESIAN_POINT('Ctrl Pts',(19.7450262601731,-17.0888130303627,-6.5749332184549));
#85902=CARTESIAN_POINT('Ctrl Pts',(19.8398772852943,-17.1434989358135,-6.58082003201506));
#85903=CARTESIAN_POINT('Ctrl Pts',(19.9655506949163,-17.2295540709509,-6.58911246717644));
#85904=CARTESIAN_POINT('Ctrl Pts',(20.0002722973563,-17.2549168048054,-6.59146243015674));
#85905=CARTESIAN_POINT('Ctrl Pts',(20.0938164011725,-17.3277168677431,-6.59802434544196));
#85906=CARTESIAN_POINT('Ctrl Pts',(20.1509032086612,-17.3772685741599,-6.60229309621258));
#85907=CARTESIAN_POINT('Ctrl Pts',(20.2120398064826,-17.4363557617218,-6.60733214526215));
#85908=CARTESIAN_POINT('Ctrl Pts',(20.2188215667602,-17.4429989947439,-6.60789802427315));
#85909=CARTESIAN_POINT('Ctrl Pts',(20.2288085650317,-17.4529145014359,-6.6087420805178));
#85910=CARTESIAN_POINT('Ctrl Pts',(20.2320483415413,-17.4561520319236,-6.60901758768075));
#85911=CARTESIAN_POINT('Ctrl Pts',(20.2377958635765,-17.461932968475,-6.60950943563549));
#85912=CARTESIAN_POINT('Ctrl Pts',(20.2403077037108,-17.4644722324413,-6.60972544767004));
#85913=CARTESIAN_POINT('Ctrl Pts',(20.2456965333109,-17.4699475420651,-6.61019117452609));
#85914=CARTESIAN_POINT('Ctrl Pts',(20.2485713590113,-17.4728855707912,-6.61044104511615));
#85915=CARTESIAN_POINT('Ctrl Pts',(20.2564885156772,-17.4810240688811,-6.61113305068991));
#85916=CARTESIAN_POINT('Ctrl Pts',(20.2615126845736,-17.4862420168139,-6.61157655820772));
#85917=CARTESIAN_POINT('Ctrl Pts',(20.2889780146913,-17.5150612389209,-6.61402464833719));
#85918=CARTESIAN_POINT('Ctrl Pts',(20.3108977326246,-17.5391507864432,-6.61606564154915));
#85919=CARTESIAN_POINT('Ctrl Pts',(20.4389307853874,-17.6865498752673,-6.62847231391311));
#85920=CARTESIAN_POINT('Ctrl Pts',(20.5310957263475,-17.8212480883874,-6.63942740376185));
#85921=CARTESIAN_POINT('Ctrl Pts',(20.6613734837904,-18.0685052257101,-6.65768271117041));
#85922=CARTESIAN_POINT('Ctrl Pts',(20.7071815180421,-18.1761816814899,-6.66512286935745));
#85923=CARTESIAN_POINT('Ctrl Pts',(20.7483642117033,-18.3006705870517,-6.67312929184691));
#85924=CARTESIAN_POINT('Ctrl Pts',(20.7527147041259,-18.3142820838135,-6.67399725963603));
#85925=CARTESIAN_POINT('Ctrl Pts',(20.7594193991405,-18.3360156367872,-6.67537155768294));
#85926=CARTESIAN_POINT('Ctrl Pts',(20.761863274625,-18.3441093677281,-6.67588081593857));
#85927=CARTESIAN_POINT('Ctrl Pts',(20.7660879237178,-18.3584097714617,-6.67677619136306));
#85928=CARTESIAN_POINT('Ctrl Pts',(20.7678888984241,-18.3646103172207,-6.67716296464597));
#85929=CARTESIAN_POINT('Ctrl Pts',(20.7715552243087,-18.3774520983253,-6.67796103397983));
#85930=CARTESIAN_POINT('Ctrl Pts',(20.7734165414381,-18.3840944130696,-6.67837219464344));
#85931=CARTESIAN_POINT('Ctrl Pts',(20.7781109607767,-18.401167712871,-6.67942490960676));
#85932=CARTESIAN_POINT('Ctrl Pts',(20.7808967256453,-18.411611593747,-6.68006492257538));
#85933=CARTESIAN_POINT('Ctrl Pts',(20.792189773325,-18.4552900830122,-6.68272562812138));
#85934=CARTESIAN_POINT('Ctrl Pts',(20.799968855721,-18.4887087649703,-6.68472279105532));
#85935=CARTESIAN_POINT('Ctrl Pts',(20.8181178077119,-18.5762624915677,-6.68986697858525));
#85936=CARTESIAN_POINT('Ctrl Pts',(20.8271923810118,-18.6306403678502,-6.69297461198297));
#85937=CARTESIAN_POINT('Ctrl Pts',(20.8479099951558,-18.7937899655436,-6.70211915236943));
#85938=CARTESIAN_POINT('Ctrl Pts',(20.8532599530273,-18.9031735973118,-6.7080073304072));
#85939=CARTESIAN_POINT('Ctrl Pts',(20.8488261989703,-19.0583049349306,-6.71645678498698));
#85940=CARTESIAN_POINT('Ctrl Pts',(20.8460284135255,-19.1040734431599,-6.7189634204485));
#85941=CARTESIAN_POINT('Ctrl Pts',(20.8396437483876,-19.1721378598308,-6.72275446854813));
#85942=CARTESIAN_POINT('Ctrl Pts',(20.8371826061535,-19.1945265915747,-6.7240117960614));
#85943=CARTESIAN_POINT('Ctrl Pts',(20.8336953902407,-19.2221793715007,-6.72558200638612));
#85944=CARTESIAN_POINT('Ctrl Pts',(20.8330058781557,-19.2274849310746,-6.7258840615606));
#85945=CARTESIAN_POINT('Ctrl Pts',(20.8261524201063,-19.2787000705403,-6.72880793340792));
#85946=CARTESIAN_POINT('Ctrl Pts',(20.8185038207325,-19.3243947000182,-6.73147945934883));
#85947=CARTESIAN_POINT('Ctrl Pts',(20.8078531538595,-19.3773006817515,-6.73468418036458));
#85948=CARTESIAN_POINT('Ctrl Pts',(20.8063020886773,-19.3847951281276,-6.73514078170952));
#85949=CARTESIAN_POINT('Ctrl Pts',(20.8037502742127,-19.3967967144346,-6.73587644755099));
#85950=CARTESIAN_POINT('Ctrl Pts',(20.8027753421833,-19.4013093560399,-6.73615407551326));
#85951=CARTESIAN_POINT('Ctrl Pts',(20.8010173005514,-19.4093197203138,-6.73664875337252));
#85952=CARTESIAN_POINT('Ctrl Pts',(20.8002400606021,-19.4128186835999,-6.73686546489816));
#85953=CARTESIAN_POINT('Ctrl Pts',(20.7985678437899,-19.4202573437952,-6.73732755458454));
#85954=CARTESIAN_POINT('Ctrl Pts',(20.7976704883132,-19.4241963962834,-6.73757306186803));
#85955=CARTESIAN_POINT('Ctrl Pts',(20.7952045667922,-19.434879568505,-6.73824106936624));
#85956=CARTESIAN_POINT('Ctrl Pts',(20.7936141955909,-19.4416185312106,-6.73866479230366));
#85957=CARTESIAN_POINT('Ctrl Pts',(20.7853698201212,-19.4758018039151,-6.74082560372004));
#85958=CARTESIAN_POINT('Ctrl Pts',(20.7782005526269,-19.5031174002884,-6.74258992917926));
#85959=CARTESIAN_POINT('Ctrl Pts',(20.7555787912444,-19.5827828712908,-6.74783025951389));
#85960=CARTESIAN_POINT('Ctrl Pts',(20.7386462105632,-19.6346863091383,-6.751365347766));
#85961=CARTESIAN_POINT('Ctrl Pts',(20.671155970708,-19.8173026057757,-6.76411145275841));
#85962=CARTESIAN_POINT('Ctrl Pts',(20.6096497610116,-19.9435970764842,-6.77347616543825));
#85963=CARTESIAN_POINT('Ctrl Pts',(20.4885706906434,-20.1400150092137,-6.7883760665901));
#85964=CARTESIAN_POINT('Ctrl Pts',(20.4361200889915,-20.2140178041928,-6.79408742514634));
#85965=CARTESIAN_POINT('Ctrl Pts',(20.3704386939896,-20.2951105509674,-6.80045471507318));
#85966=CARTESIAN_POINT('Ctrl Pts',(20.3616923828878,-20.3056968168467,-6.80128835463687));
#85967=CARTESIAN_POINT('Ctrl Pts',(20.3475003789504,-20.3225379522307,-6.80261866491772));
#85968=CARTESIAN_POINT('Ctrl Pts',(20.3421199696312,-20.328847093074,-6.80311797911128));
#85969=CARTESIAN_POINT('Ctrl Pts',(20.3325008427541,-20.3399933051705,-6.804001853058));
#85970=CARTESIAN_POINT('Ctrl Pts',(20.328276914794,-20.3448429487397,-6.8043870158259));
#85971=CARTESIAN_POINT('Ctrl Pts',(20.3194300644443,-20.3549073646952,-6.80518762348243));
#85972=CARTESIAN_POINT('Ctrl Pts',(20.3148033545621,-20.3601187162842,-6.80560290389716));
#85973=CARTESIAN_POINT('Ctrl Pts',(20.3027209612745,-20.3735932645148,-6.80667862059588));
#85974=CARTESIAN_POINT('Ctrl Pts',(20.2952256381819,-20.3818207502664,-6.80733738131728));
#85975=CARTESIAN_POINT('Ctrl Pts',(20.2623925116868,-20.4172950871922,-6.81018673204135));
#85976=CARTESIAN_POINT('Ctrl Pts',(20.2364028401232,-20.4439314049518,-6.81234932037613));
#85977=CARTESIAN_POINT('Ctrl Pts',(20.1654924194756,-20.5128728535719,-6.81802520626901));
#85978=CARTESIAN_POINT('Ctrl Pts',(20.1194009337238,-20.5539237560652,-6.82148754409593));
#85979=CARTESIAN_POINT('Ctrl Pts',(19.9574244261251,-20.6859584487774,-6.83304903405252));
#85980=CARTESIAN_POINT('Ctrl Pts',(19.833878030955,-20.7668400265856,-6.84085978024349));
#85981=CARTESIAN_POINT('Ctrl Pts',(19.6401114313903,-20.8665874515746,-6.85296096597903));
#85982=CARTESIAN_POINT('Ctrl Pts',(19.5757058648517,-20.8957623601569,-6.85696745378742));
#85983=CARTESIAN_POINT('Ctrl Pts',(19.5012534312635,-20.9250937493032,-6.86171120454358));
#85984=CARTESIAN_POINT('Ctrl Pts',(19.4925143219775,-20.9284697790188,-6.86226973542677));
#85985=CARTESIAN_POINT('Ctrl Pts',(19.4794929660384,-20.9334010171762,-6.86310490313351));
#85986=CARTESIAN_POINT('Ctrl Pts',(19.4752275058808,-20.9350006396658,-6.86337895091229));
#85987=CARTESIAN_POINT('Ctrl Pts',(19.4676106768614,-20.9378290753481,-6.86386920826725));
#85988=CARTESIAN_POINT('Ctrl Pts',(19.4642613321553,-20.9390631918023,-6.86408509736251));
#85989=CARTESIAN_POINT('Ctrl Pts',(19.4570325280633,-20.9417060077999,-6.86455172454537));
#85990=CARTESIAN_POINT('Ctrl Pts',(19.4531521212957,-20.9431118150111,-6.86480262458211));
#85991=CARTESIAN_POINT('Ctrl Pts',(19.4423785923912,-20.9469792843731,-6.86550032297558));
#85992=CARTESIAN_POINT('Ctrl Pts',(19.4354768536649,-20.9494165302727,-6.8659485305063));
#85993=CARTESIAN_POINT('Ctrl Pts',(19.3967263510014,-20.9628750832011,-6.86847146220071));
#85994=CARTESIAN_POINT('Ctrl Pts',(19.3646324932815,-20.9731697548409,-6.87058521452178));
#85995=CARTESIAN_POINT('Ctrl Pts',(19.2634050235159,-21.0029946847435,-6.87729822382512));
#85996=CARTESIAN_POINT('Ctrl Pts',(19.193517172832,-21.019774507139,-6.88199781431464));
#85997=CARTESIAN_POINT('Ctrl Pts',(19.0984184415285,-21.0375477351631,-6.88837432458532));
#85998=CARTESIAN_POINT('Ctrl Pts',(19.0738408090841,-21.0416933667544,-6.89002084513981));
#85999=CARTESIAN_POINT('Ctrl Pts',(18.8813730648572,-21.070672500803,-6.90288308672149));
#86000=CARTESIAN_POINT('Ctrl Pts',(18.7110874713322,-21.0756733060515,-6.91400215221685));
#86001=CARTESIAN_POINT('Ctrl Pts',(18.5187396621086,-21.0581571597103,-6.92589487591079));
#86002=CARTESIAN_POINT('Ctrl Pts',(18.4955054126994,-21.0556528694072,-6.92732166519893));
#86003=CARTESIAN_POINT('Ctrl Pts',(18.4627821770708,-21.0515766737402,-6.92931807621384));
#86004=CARTESIAN_POINT('Ctrl Pts',(18.4532557976113,-21.0503240965053,-6.92989770396659));
#86005=CARTESIAN_POINT('Ctrl Pts',(18.4378165229655,-21.0481870349397,-6.93083463906088));
#86006=CARTESIAN_POINT('Ctrl Pts',(18.4318983464809,-21.0473422941367,-6.93119319731217));
#86007=CARTESIAN_POINT('Ctrl Pts',(18.419538173269,-21.0455245887953,-6.93194085185123));
#86008=CARTESIAN_POINT('Ctrl Pts',(18.4130969217915,-21.0445469314263,-6.93232979539597));
#86009=CARTESIAN_POINT('Ctrl Pts',(18.3978212427824,-21.0421561866463,-6.93325062082878));
#86010=CARTESIAN_POINT('Ctrl Pts',(18.3889910124291,-21.0407167935406,-6.93378166330591));
#86011=CARTESIAN_POINT('Ctrl Pts',(18.3594461566719,-21.0357082908153,-6.93555447949112));
#86012=CARTESIAN_POINT('Ctrl Pts',(18.3387751956277,-21.0318865891334,-6.93678823401119));
#86013=CARTESIAN_POINT('Ctrl Pts',(18.2276664622002,-21.0096282047749,-6.94338915930166));
#86014=CARTESIAN_POINT('Ctrl Pts',(18.1384457872673,-20.985599151113,-6.94857382998983));
#86015=CARTESIAN_POINT('Ctrl Pts',(17.9186476997537,-20.910688874738,-6.96136637431337));
#86016=CARTESIAN_POINT('Ctrl Pts',(17.7910330296627,-20.8525450690877,-6.96880102409604));
#86017=CARTESIAN_POINT('Ctrl Pts',(17.6108382003692,-20.7477989591045,-6.98039040851198));
#86018=CARTESIAN_POINT('Ctrl Pts',(17.5532984805687,-20.7105017086431,-6.98428168865104));
#86019=CARTESIAN_POINT('Ctrl Pts',(17.490106209662,-20.6650394551776,-6.98889687856186));
#86020=CARTESIAN_POINT('Ctrl Pts',(17.4825736368637,-20.6595444319488,-6.98945278129145));
#86021=CARTESIAN_POINT('Ctrl Pts',(17.4714223380889,-20.6512961249973,-6.99028476773022));
#86022=CARTESIAN_POINT('Ctrl Pts',(17.4677756695544,-20.6485805659885,-6.99055829108771));
#86023=CARTESIAN_POINT('Ctrl Pts',(17.4614195361621,-20.6438154464929,-6.99103763440959));
#86024=CARTESIAN_POINT('Ctrl Pts',(17.4587062239407,-20.6417710870099,-6.9912430892678));
#86025=CARTESIAN_POINT('Ctrl Pts',(17.452819062595,-20.6373131174907,-6.99169069856052));
#86026=CARTESIAN_POINT('Ctrl Pts',(17.4496471545203,-20.634897105012,-6.9919330186152));
#86027=CARTESIAN_POINT('Ctrl Pts',(17.4411877201961,-20.6284157879533,-6.99258233414978));
#86028=CARTESIAN_POINT('Ctrl Pts',(17.4359125995587,-20.6243344710283,-6.992990434723));
#86029=CARTESIAN_POINT('Ctrl Pts',(17.4241749041285,-20.6151641174227,-6.99390550907587));
#86030=CARTESIAN_POINT('Ctrl Pts',(17.417722560256,-20.6100622304418,-6.99441332646983));
#86031=CARTESIAN_POINT('Ctrl Pts',(17.3981791753551,-20.594423249501,-6.99596566560015));
#86032=CARTESIAN_POINT('Ctrl Pts',(17.3851840346272,-20.5837680166732,-6.99701746916403));
#86033=CARTESIAN_POINT('Ctrl Pts',(17.3368453813657,-20.5431612695802,-7.00099987075799));
#86034=CARTESIAN_POINT('Ctrl Pts',(17.3023630944086,-20.5122084572404,-7.00398343556874));
#86035=CARTESIAN_POINT('Ctrl Pts',(17.2194705806093,-20.4327375201702,-7.01146386641024));
#86036=CARTESIAN_POINT('Ctrl Pts',(17.1723471433782,-20.3829517215942,-7.01599584036224));
#86037=CARTESIAN_POINT('Ctrl Pts',(17.0230827516861,-20.2090827754921,-7.03113752218766));
#86038=CARTESIAN_POINT('Ctrl Pts',(16.9326383657498,-20.0756589440136,-7.04162667761467));
#86039=CARTESIAN_POINT('Ctrl Pts',(16.8471281735806,-19.9121923280529,-7.05299063890773));
#86040=CARTESIAN_POINT('Ctrl Pts',(16.836460239165,-19.8909342493639,-7.05444320153705));
#86041=CARTESIAN_POINT('Ctrl Pts',(16.8219582091015,-19.8607787657603,-7.05646922583326));
#86042=CARTESIAN_POINT('Ctrl Pts',(16.8178237869933,-19.852028544443,-7.05705309541346));
#86043=CARTESIAN_POINT('Ctrl Pts',(16.8112273404217,-19.8378161149772,-7.05799503237767));
#86044=CARTESIAN_POINT('Ctrl Pts',(16.8087282806853,-19.8323713409289,-7.05835437694544));
#86045=CARTESIAN_POINT('Ctrl Pts',(16.8035640625956,-19.8209927520846,-7.05910222649855));
#86046=CARTESIAN_POINT('Ctrl Pts',(16.8009030694787,-19.8150571071859,-7.0594905850705));
#86047=CARTESIAN_POINT('Ctrl Pts',(16.7946705099276,-19.8009812399099,-7.0604074415907));
#86048=CARTESIAN_POINT('Ctrl Pts',(16.7911227548355,-19.7928305600283,-7.06093511992045));
#86049=CARTESIAN_POINT('Ctrl Pts',(16.7794904341133,-19.7656395036212,-7.06268495435289));
#86050=CARTESIAN_POINT('Ctrl Pts',(16.7716334439858,-19.7465026303007,-7.06389937726305));
#86051=CARTESIAN_POINT('Ctrl Pts',(16.7576410919479,-19.7109476353391,-7.066125921824));
#86052=CARTESIAN_POINT('Ctrl Pts',(16.7514278355577,-19.6945654719617,-7.06714032154971));
#86053=CARTESIAN_POINT('Ctrl Pts',(16.7454194581678,-19.6781104796424,-7.06814844662885));
#86054=CARTESIAN_POINT('Ctrl Pts',(16.7454194485728,-19.6781104533646,-6.84500598787601));
#86055=CARTESIAN_POINT('Ctrl Pts',(16.7536780380464,-19.7007280459546,-6.84341661262277));
#86056=CARTESIAN_POINT('Ctrl Pts',(16.7623223866146,-19.7232044385535,-6.841824850225));
#86057=CARTESIAN_POINT('Ctrl Pts',(16.7857100470872,-19.7810495514162,-6.8377020043978));
#86058=CARTESIAN_POINT('Ctrl Pts',(16.8010330336016,-19.8161734120292,-6.83517284233548));
#86059=CARTESIAN_POINT('Ctrl Pts',(16.8576523309627,-19.936906172792,-6.82641396455609));
#86060=CARTESIAN_POINT('Ctrl Pts',(16.9037554382877,-20.0201428847521,-6.82026484169948));
#86061=CARTESIAN_POINT('Ctrl Pts',(16.9803711804393,-20.1388496765648,-6.8113990453225));
#86062=CARTESIAN_POINT('Ctrl Pts',(17.006707645613,-20.1768623756601,-6.8085426759325));
#86063=CARTESIAN_POINT('Ctrl Pts',(17.0414157734736,-20.2236097468993,-6.80500496816375));
#86064=CARTESIAN_POINT('Ctrl Pts',(17.0486437955743,-20.2331741434187,-6.80427976861819));
#86065=CARTESIAN_POINT('Ctrl Pts',(17.0603174042016,-20.2483513486212,-6.80312660074575));
#86066=CARTESIAN_POINT('Ctrl Pts',(17.0647108159088,-20.2540037912338,-6.80269658935759));
#86067=CARTESIAN_POINT('Ctrl Pts',(17.073076928698,-20.2646554471408,-6.80188519529132));
#86068=CARTESIAN_POINT('Ctrl Pts',(17.0770437308944,-20.2696591726785,-6.8015035845218));
#86069=CARTESIAN_POINT('Ctrl Pts',(17.0860738390126,-20.2809444913788,-6.80064184084566));
#86070=CARTESIAN_POINT('Ctrl Pts',(17.0911505562668,-20.2872152639977,-6.80016225264278));
#86071=CARTESIAN_POINT('Ctrl Pts',(17.1062386150198,-20.3056357371196,-6.79875109607873));
#86072=CARTESIAN_POINT('Ctrl Pts',(17.1163499098169,-20.3177031306008,-6.7978235817372));
#86073=CARTESIAN_POINT('Ctrl Pts',(17.2076554603322,-20.4242354574733,-6.78960463271056));
#86074=CARTESIAN_POINT('Ctrl Pts',(17.2969092350462,-20.5114810165515,-6.78267609119741));
#86075=CARTESIAN_POINT('Ctrl Pts',(17.5230065109461,-20.6964942362747,-6.76672052178679));
#86076=CARTESIAN_POINT('Ctrl Pts',(17.6648044211286,-20.786821714059,-6.75786060465836));
#86077=CARTESIAN_POINT('Ctrl Pts',(17.8351458866485,-20.8688239784094,-6.74686255675113));
#86078=CARTESIAN_POINT('Ctrl Pts',(17.8546927905106,-20.8778690587652,-6.74559503727467));
#86079=CARTESIAN_POINT('Ctrl Pts',(17.8801233784215,-20.8891688890996,-6.74393467957359));
#86080=CARTESIAN_POINT('Ctrl Pts',(17.8858846193461,-20.8916981436783,-6.74355778715657));
#86081=CARTESIAN_POINT('Ctrl Pts',(17.894742296601,-20.8955397647392,-6.74297706638763));
#86082=CARTESIAN_POINT('Ctrl Pts',(17.8978307860735,-20.8968705240081,-6.74277434619168));
#86083=CARTESIAN_POINT('Ctrl Pts',(17.9042045628944,-20.8995988495985,-6.74235547880888));
#86084=CARTESIAN_POINT('Ctrl Pts',(17.9074901901533,-20.9009954540692,-6.74213927397251));
#86085=CARTESIAN_POINT('Ctrl Pts',(17.9149829906281,-20.9041580256838,-6.74164558926162));
#86086=CARTESIAN_POINT('Ctrl Pts',(17.9191923337179,-20.9059186996775,-6.74136779393161));
#86087=CARTESIAN_POINT('Ctrl Pts',(17.9301582013881,-20.9104638794813,-6.74064299419499));
#86088=CARTESIAN_POINT('Ctrl Pts',(17.936923444624,-20.9132270051557,-6.74019474783167));
#86089=CARTESIAN_POINT('Ctrl Pts',(17.9802287930293,-20.9306531162098,-6.73731912937884));
#86090=CARTESIAN_POINT('Ctrl Pts',(18.0171551799489,-20.9443283453943,-6.7348385062367));
#86091=CARTESIAN_POINT('Ctrl Pts',(18.2352222370377,-21.0182398469808,-6.72011010559865));
#86092=CARTESIAN_POINT('Ctrl Pts',(18.423466191539,-21.0547853843035,-6.70717970967866));
#86093=CARTESIAN_POINT('Ctrl Pts',(18.6690805391439,-21.068721482032,-6.69136694511972));
#86094=CARTESIAN_POINT('Ctrl Pts',(18.7241904573857,-21.0696942561511,-6.6878781972971));
#86095=CARTESIAN_POINT('Ctrl Pts',(18.8135720992245,-21.0677820782871,-6.68232117486196));
#86096=CARTESIAN_POINT('Ctrl Pts',(18.847843278002,-21.0662150898382,-6.6802144709364));
#86097=CARTESIAN_POINT('Ctrl Pts',(18.8928445504151,-21.063059976504,-6.67747811850878));
#86098=CARTESIAN_POINT('Ctrl Pts',(18.9036204154534,-21.0622214900432,-6.67682513244238));
#86099=CARTESIAN_POINT('Ctrl Pts',(18.921262400303,-21.0607127293788,-6.67575965511964));
#86100=CARTESIAN_POINT('Ctrl Pts',(18.9281324035724,-21.0600913626422,-6.67534563454353));
#86101=CARTESIAN_POINT('Ctrl Pts',(18.9414269063701,-21.0588233832749,-6.67454612194857));
#86102=CARTESIAN_POINT('Ctrl Pts',(18.9478517176283,-21.0581809357444,-6.67416050361428));
#86103=CARTESIAN_POINT('Ctrl Pts',(18.962682446802,-21.0566293787908,-6.6732720724199));
#86104=CARTESIAN_POINT('Ctrl Pts',(18.9710860947131,-21.0556992823124,-6.67276992567742));
#86105=CARTESIAN_POINT('Ctrl Pts',(18.9936779611847,-21.0530617720149,-6.67142327440938));
#86106=CARTESIAN_POINT('Ctrl Pts',(19.0078549910934,-21.0512609823728,-6.67058171157713));
#86107=CARTESIAN_POINT('Ctrl Pts',(19.1378034867022,-21.0334158707581,-6.66289745615126));
#86108=CARTESIAN_POINT('Ctrl Pts',(19.2520854550784,-21.0079528232304,-6.65637168629916));
#86109=CARTESIAN_POINT('Ctrl Pts',(19.5192312097798,-20.924724214512,-6.64105381461462));
#86110=CARTESIAN_POINT('Ctrl Pts',(19.6686357511708,-20.858481829157,-6.63244527751377));
#86111=CARTESIAN_POINT('Ctrl Pts',(19.83678700674,-20.7593720929295,-6.62123557181563));
#86112=CARTESIAN_POINT('Ctrl Pts',(19.8642425563889,-20.7423308552909,-6.61935069636158));
#86113=CARTESIAN_POINT('Ctrl Pts',(19.8973464684706,-20.7207188050917,-6.61699672473154));
#86114=CARTESIAN_POINT('Ctrl Pts',(19.9033769143353,-20.7167376139198,-6.6165645336402));
#86115=CARTESIAN_POINT('Ctrl Pts',(19.9128023656273,-20.7104455772289,-6.61588352173284));
#86116=CARTESIAN_POINT('Ctrl Pts',(19.9162112955816,-20.7081555504069,-6.61563608014102));
#86117=CARTESIAN_POINT('Ctrl Pts',(19.9225730850745,-20.7038549549787,-6.61517212623207));
#86118=CARTESIAN_POINT('Ctrl Pts',(19.9255275261901,-20.7018468263021,-6.61495577818221));
#86119=CARTESIAN_POINT('Ctrl Pts',(19.9322631359734,-20.6972436759095,-6.61446052475571));
#86120=CARTESIAN_POINT('Ctrl Pts',(19.936040951097,-20.6946438483829,-6.61418129597108));
#86121=CARTESIAN_POINT('Ctrl Pts',(19.9476376019537,-20.6866075811814,-6.61331974459068));
#86122=CARTESIAN_POINT('Ctrl Pts',(19.9554280999317,-20.6811307291466,-6.61273476808163));
#86123=CARTESIAN_POINT('Ctrl Pts',(20.059666091297,-20.6067937251717,-6.60482693076226));
#86124=CARTESIAN_POINT('Ctrl Pts',(20.1501920635098,-20.5300134226837,-6.59703559225824));
#86125=CARTESIAN_POINT('Ctrl Pts',(20.3109865785519,-20.3686018886004,-6.5819853909188));
#86126=CARTESIAN_POINT('Ctrl Pts',(20.3820512515836,-20.2852584589575,-6.57475458099747));
#86127=CARTESIAN_POINT('Ctrl Pts',(20.4787413927651,-20.1522495563294,-6.5641851107618));
#86128=CARTESIAN_POINT('Ctrl Pts',(20.5093731491009,-20.1064576762435,-6.56069805937811));
#86129=CARTESIAN_POINT('Ctrl Pts',(20.5561247201943,-20.0302978367596,-6.55514342264989));
#86130=CARTESIAN_POINT('Ctrl Pts',(20.5733512388232,-20.0006429120504,-6.55303744911663));
#86131=CARTESIAN_POINT('Ctrl Pts',(20.5950502021521,-19.9611074926157,-6.55030189220939));
#86132=CARTESIAN_POINT('Ctrl Pts',(20.6001772741398,-19.9515940050091,-6.54964898823839));
#86133=CARTESIAN_POINT('Ctrl Pts',(20.6084571200258,-19.9359446543029,-6.5485836105344));
#86134=CARTESIAN_POINT('Ctrl Pts',(20.6116531038736,-19.9298319900741,-6.54816960803367));
#86135=CARTESIAN_POINT('Ctrl Pts',(20.6177828965845,-19.9179672302272,-6.54737010662314));
#86136=CARTESIAN_POINT('Ctrl Pts',(20.6207203728542,-19.9122171251438,-6.54698448152206));
#86137=CARTESIAN_POINT('Ctrl Pts',(20.6274437087045,-19.8989062349463,-6.54609600083667));
#86138=CARTESIAN_POINT('Ctrl Pts',(20.6312106859756,-19.8913359952631,-6.54559381160812));
#86139=CARTESIAN_POINT('Ctrl Pts',(20.6412228700802,-19.8709092494572,-6.54424697115701));
#86140=CARTESIAN_POINT('Ctrl Pts',(20.6473834685256,-19.8580115905372,-6.54340526293642));
#86141=CARTESIAN_POINT('Ctrl Pts',(20.702798841186,-19.7389088314875,-6.53570959171701));
#86142=CARTESIAN_POINT('Ctrl Pts',(20.7432983510267,-19.6288454834824,-6.5291736803899));
#86143=CARTESIAN_POINT('Ctrl Pts',(20.8180594019977,-19.3583604642705,-6.51381210631146));
#86144=CARTESIAN_POINT('Ctrl Pts',(20.8432101515545,-19.1962391289494,-6.5051718396048));
#86145=CARTESIAN_POINT('Ctrl Pts',(20.8506615694375,-19.001299386526,-6.4939590367058));
#86146=CARTESIAN_POINT('Ctrl Pts',(20.8511614324631,-18.9697160099649,-6.49211550114772));
#86147=CARTESIAN_POINT('Ctrl Pts',(20.8509076035842,-18.930959910016,-6.48980754471176));
#86148=CARTESIAN_POINT('Ctrl Pts',(20.8508241299618,-18.9237849870449,-6.48937834739955));
#86149=CARTESIAN_POINT('Ctrl Pts',(20.8506357189086,-18.912515734333,-6.48870101438323));
#86150=CARTESIAN_POINT('Ctrl Pts',(20.8505553716861,-18.908420971466,-6.48845423338577));
#86151=CARTESIAN_POINT('Ctrl Pts',(20.850382658026,-18.9007533541636,-6.48799083316416));
#86152=CARTESIAN_POINT('Ctrl Pts',(20.8502931259038,-18.8971804917463,-6.4877743740464));
#86153=CARTESIAN_POINT('Ctrl Pts',(20.8500675816192,-18.889006518436,-6.48727795831878));
#86154=CARTESIAN_POINT('Ctrl Pts',(20.8499256103671,-18.8844056276888,-6.4869976724417));
#86155=CARTESIAN_POINT('Ctrl Pts',(20.8495148649811,-18.8723681505808,-6.48626214392911));
#86156=CARTESIAN_POINT('Ctrl Pts',(20.8492218860273,-18.8649325288807,-6.48580559954916));
#86157=CARTESIAN_POINT('Ctrl Pts',(20.8470114327017,-18.8154637210862,-6.48275425591465));
#86158=CARTESIAN_POINT('Ctrl Pts',(20.843880486483,-18.7734971799336,-6.48009862150874));
#86159=CARTESIAN_POINT('Ctrl Pts',(20.8387360564558,-18.7243396469215,-6.4769301205581));
#86160=CARTESIAN_POINT('Ctrl Pts',(20.8379323540438,-18.7170281909219,-6.47645733971364));
#86161=CARTESIAN_POINT('Ctrl Pts',(20.836257315014,-18.7024880906132,-6.47551429942186));
#86162=CARTESIAN_POINT('Ctrl Pts',(20.8353867557889,-18.6952594460115,-6.47504406866501));
#86163=CARTESIAN_POINT('Ctrl Pts',(20.8135700365253,-18.521654434538,-6.46371936701003));
#86164=CARTESIAN_POINT('Ctrl Pts',(20.772967309756,-18.3583428964865,-6.45243220453915));
#86165=CARTESIAN_POINT('Ctrl Pts',(20.6927190443868,-18.1466743416921,-6.4378410200488));
#86166=CARTESIAN_POINT('Ctrl Pts',(20.669653004821,-18.0927106810954,-6.43411766848078));
#86167=CARTESIAN_POINT('Ctrl Pts',(20.6289083289105,-18.0073839390058,-6.42823248200722));
#86168=CARTESIAN_POINT('Ctrl Pts',(20.6126214110876,-17.9753941844382,-6.4260263188917));
#86169=CARTESIAN_POINT('Ctrl Pts',(20.5902959339706,-17.9341713713622,-6.42318193770447));
#86170=CARTESIAN_POINT('Ctrl Pts',(20.5849885013125,-17.9245510782099,-6.42251801616075));
#86171=CARTESIAN_POINT('Ctrl Pts',(20.5762080643467,-17.9089244642064,-6.42143926542278));
#86172=CARTESIAN_POINT('Ctrl Pts',(20.5727800545382,-17.9028932187188,-6.4210228327517));
#86173=CARTESIAN_POINT('Ctrl Pts',(20.5661117969379,-17.8912941686638,-6.42022177229258));
#86174=CARTESIAN_POINT('Ctrl Pts',(20.5628756651789,-17.8857240976922,-6.41983700183805));
#86175=CARTESIAN_POINT('Ctrl Pts',(20.5553807169491,-17.8729582033306,-6.41895491142425));
#86176=CARTESIAN_POINT('Ctrl Pts',(20.5511045742551,-17.8657726369144,-6.41845822704092));
#86177=CARTESIAN_POINT('Ctrl Pts',(20.5395707938467,-17.8466501619912,-6.41713582273701));
#86178=CARTESIAN_POINT('Ctrl Pts',(20.5322373087074,-17.8347593135334,-6.41631287917404));
#86179=CARTESIAN_POINT('Ctrl Pts',(20.4714672711647,-17.7383726474511,-6.40963480348134));
#86180=CARTESIAN_POINT('Ctrl Pts',(20.4122211229211,-17.6576810987769,-6.40400641677406));
#86181=CARTESIAN_POINT('Ctrl Pts',(20.2361676815161,-17.4504181774575,-6.38902092584685));
#86182=CARTESIAN_POINT('Ctrl Pts',(20.1093107176857,-17.333431345525,-6.3799835453606));
#86183=CARTESIAN_POINT('Ctrl Pts',(19.9372894117595,-17.2097660651834,-6.36791346258814));
#86184=CARTESIAN_POINT('Ctrl Pts',(19.9042057592057,-17.1873746832272,-6.36559693712837));
#86185=CARTESIAN_POINT('Ctrl Pts',(19.8640243073331,-17.161806384331,-6.3627640027438));
#86186=CARTESIAN_POINT('Ctrl Pts',(19.8575151603805,-17.1577141261671,-6.36230449109463));
#86187=CARTESIAN_POINT('Ctrl Pts',(19.8474097087719,-17.1514374422352,-6.36158994975569));
#86188=CARTESIAN_POINT('Ctrl Pts',(19.8438288633841,-17.1492280795106,-6.36133653180358));
#86189=CARTESIAN_POINT('Ctrl Pts',(19.8372045956612,-17.1451681574711,-6.36086727512391));
#86190=CARTESIAN_POINT('Ctrl Pts',(19.8341630800822,-17.1433145979101,-6.3606516373507));
#86191=CARTESIAN_POINT('Ctrl Pts',(19.8273127401953,-17.139163538103,-6.36016556006592));
#86192=CARTESIAN_POINT('Ctrl Pts',(19.8235013693966,-17.1368703763357,-6.35989484456079));
#86193=CARTESIAN_POINT('Ctrl Pts',(19.8137318520794,-17.1310342727399,-6.35920029081883));
#86194=CARTESIAN_POINT('Ctrl Pts',(19.8077635324534,-17.1275085844041,-6.35877537223765));
#86195=CARTESIAN_POINT('Ctrl Pts',(19.7728196821254,-17.1070969160525,-6.35628447796757));
#86196=CARTESIAN_POINT('Ctrl Pts',(19.7434652212802,-17.0908730841479,-6.35417989372362));
#86197=CARTESIAN_POINT('Ctrl Pts',(19.6975171370094,-17.0668849815665,-6.35088133063223));
#86198=CARTESIAN_POINT('Ctrl Pts',(19.6811857390117,-17.058626543587,-6.3497080907537));
#86199=CARTESIAN_POINT('Ctrl Pts',(19.6425621221851,-17.0397201767748,-6.34693475346956));
#86200=CARTESIAN_POINT('Ctrl Pts',(19.6201866386643,-17.0292487349793,-6.34532916368714));
#86201=CARTESIAN_POINT('Ctrl Pts',(19.55662327483,-17.0008471136649,-6.34078012479797));
#86202=CARTESIAN_POINT('Ctrl Pts',(19.5150409357475,-16.9838329553595,-6.33781844973897));
#86203=CARTESIAN_POINT('Ctrl Pts',(19.3704829489971,-16.929987468101,-6.32762833700818));
#86204=CARTESIAN_POINT('Ctrl Pts',(19.2652049020342,-16.8998133509897,-6.32039830598454));
#86205=CARTESIAN_POINT('Ctrl Pts',(19.1041214843611,-16.8668788560421,-6.30983047157207));
#86206=CARTESIAN_POINT('Ctrl Pts',(19.0497689852065,-16.8579582465252,-6.30634427169256));
#86207=CARTESIAN_POINT('Ctrl Pts',(18.9611055010472,-16.8469376707463,-6.30079083250703));
#86208=CARTESIAN_POINT('Ctrl Pts',(18.9269852355622,-16.8435358116761,-6.29868522564573));
#86209=CARTESIAN_POINT('Ctrl Pts',(18.8820200893326,-16.8401534560553,-6.29595006811836));
#86210=CARTESIAN_POINT('Ctrl Pts',(18.8712382213373,-16.8394253979084,-6.29529720537102));
#86211=CARTESIAN_POINT('Ctrl Pts',(18.8535659078902,-16.8383679201015,-6.29423187768985));
#86212=CARTESIAN_POINT('Ctrl Pts',(18.8466786886885,-16.8379895718391,-6.2938178842653));
#86213=CARTESIAN_POINT('Ctrl Pts',(18.8333408036588,-16.8373222238749,-6.29301838846832));
#86214=CARTESIAN_POINT('Ctrl Pts',(18.8268904312178,-16.8370290637167,-6.29263275996703));
#86215=CARTESIAN_POINT('Ctrl Pts',(18.8119899302758,-16.8364201568479,-6.29174425441906));
#86216=CARTESIAN_POINT('Ctrl Pts',(18.8035390133308,-16.8361255163017,-6.29124204384785));
#86217=CARTESIAN_POINT('Ctrl Pts',(18.7807983310311,-16.8354690559655,-6.28989510835804));
#86218=CARTESIAN_POINT('Ctrl Pts',(18.7665061357712,-16.8352013116727,-6.28905332709893));
#86219=CARTESIAN_POINT('Ctrl Pts',(18.6350479479026,-16.8340703656135,-6.28135182791991));
#86220=CARTESIAN_POINT('Ctrl Pts',(18.5179952719898,-16.84279050409,-6.27481073902645));
#86221=CARTESIAN_POINT('Ctrl Pts',(18.2404054660157,-16.8868348208592,-6.25942582610652));
#86222=CARTESIAN_POINT('Ctrl Pts',(18.0821083924364,-16.9312160528081,-6.25076841668036));
#86223=CARTESIAN_POINT('Ctrl Pts',(17.9016686564573,-17.0052368164309,-6.23955361745208));
#86224=CARTESIAN_POINT('Ctrl Pts',(17.8730712694035,-17.0177136079514,-6.23773208932225));
#86225=CARTESIAN_POINT('Ctrl Pts',(17.8382749432368,-17.0338194254977,-6.23544864359803));
#86226=CARTESIAN_POINT('Ctrl Pts',(17.8318034802732,-17.0368546973697,-6.23502107085787));
#86227=CARTESIAN_POINT('Ctrl Pts',(17.8216539560528,-17.0416779276029,-6.23434573451489));
#86228=CARTESIAN_POINT('Ctrl Pts',(17.8179654235865,-17.0434439022241,-6.23409931239371));
#86229=CARTESIAN_POINT('Ctrl Pts',(17.8110620452372,-17.0467736847109,-6.23363620989974));
#86230=CARTESIAN_POINT('Ctrl Pts',(17.807846035753,-17.048334952087,-6.23341968736249));
#86231=CARTESIAN_POINT('Ctrl Pts',(17.800489649668,-17.0519292902876,-6.23292262615336));
#86232=CARTESIAN_POINT('Ctrl Pts',(17.7963519651558,-17.0539677458202,-6.23264175497193));
#86233=CARTESIAN_POINT('Ctrl Pts',(17.7855282359894,-17.0593441521694,-6.231903698042));
#86234=CARTESIAN_POINT('Ctrl Pts',(17.7788532137776,-17.0627039780824,-6.23144519626959));
#86235=CARTESIAN_POINT('Ctrl Pts',(17.7341726007515,-17.0854909548363,-6.22835435169245));
#86236=CARTESIAN_POINT('Ctrl Pts',(17.6967469970419,-17.1060269547391,-6.22565941201138));
#86237=CARTESIAN_POINT('Ctrl Pts',(17.6537632245609,-17.1313327056938,-6.2224602927846));
#86238=CARTESIAN_POINT('Ctrl Pts',(17.6475745436013,-17.1350188187123,-6.22199711003756));
#86239=CARTESIAN_POINT('Ctrl Pts',(17.5067332063704,-17.2198837888335,-6.21139884073029));
#86240=CARTESIAN_POINT('Ctrl Pts',(17.3815204018575,-17.3157810046314,-6.20082558747141));
#86241=CARTESIAN_POINT('Ctrl Pts',(17.1996368741147,-17.4903510061928,-6.18444645934869));
#86242=CARTESIAN_POINT('Ctrl Pts',(17.1356824215481,-17.5605715656691,-6.17842083327181));
#86243=CARTESIAN_POINT('Ctrl Pts',(17.0633767518922,-17.6515531917824,-6.17128275493334));
#86244=CARTESIAN_POINT('Ctrl Pts',(17.0503589549969,-17.6684514726908,-6.16998270808881));
#86245=CARTESIAN_POINT('Ctrl Pts',(17.0322147355487,-17.6927554246906,-6.16814848201649));
#86246=CARTESIAN_POINT('Ctrl Pts',(17.0268770668084,-17.7000010856115,-6.16760604876475));
#86247=CARTESIAN_POINT('Ctrl Pts',(17.0177495690953,-17.7125581794175,-6.16667346187058));
#86248=CARTESIAN_POINT('Ctrl Pts',(17.0139378254468,-17.7178534587254,-6.16628246096825));
#86249=CARTESIAN_POINT('Ctrl Pts',(17.0066870510081,-17.7280250901367,-6.16553568292628));
#86250=CARTESIAN_POINT('Ctrl Pts',(17.0032440433173,-17.7328985180634,-6.16517975496167));
#86251=CARTESIAN_POINT('Ctrl Pts',(16.9943461643336,-17.745606751596,-6.16425641712621));
#86252=CARTESIAN_POINT('Ctrl Pts',(16.9889235641388,-17.7534640700907,-6.16369024335043));
#86253=CARTESIAN_POINT('Ctrl Pts',(16.9706219477666,-17.7803705493189,-6.16176718612473));
#86254=CARTESIAN_POINT('Ctrl Pts',(16.9579999313758,-17.7995931525738,-6.16041999474128));
#86255=CARTESIAN_POINT('Ctrl Pts',(16.8517988247959,-17.9672217507519,-6.1488890428652));
#86256=CARTESIAN_POINT('Ctrl Pts',(16.776691026808,-18.1265196858736,-6.13945578184607));
#86257=CARTESIAN_POINT('Ctrl Pts',(16.695013960994,-18.3759801243864,-6.12517347375519));
#86258=CARTESIAN_POINT('Ctrl Pts',(16.6730620305314,-18.460273191983,-6.12040912736751));
#86259=CARTESIAN_POINT('Ctrl Pts',(16.6490998648993,-18.58279614198,-6.11328125960133));
#86260=CARTESIAN_POINT('Ctrl Pts',(16.6428359519368,-18.6201075673872,-6.11108386664042));
#86261=CARTESIAN_POINT('Ctrl Pts',(16.6365221765187,-18.6650625222771,-6.10838291865366));
#86262=CARTESIAN_POINT('Ctrl Pts',(16.6355092976138,-18.6725664583643,-6.10793029583871));
#86263=CARTESIAN_POINT('Ctrl Pts',(16.633999500558,-18.684223237831,-6.10722420073402));
#86264=CARTESIAN_POINT('Ctrl Pts',(16.6334745843573,-18.6883724795121,-6.1069722800572));
#86265=CARTESIAN_POINT('Ctrl Pts',(16.6325251661729,-18.6960601177614,-6.10650439715054));
#86266=CARTESIAN_POINT('Ctrl Pts',(16.6320973021972,-18.6995980409812,-6.1062886268257));
#86267=CARTESIAN_POINT('Ctrl Pts',(16.6311517266855,-18.7075859865194,-6.10580045657992));
#86268=CARTESIAN_POINT('Ctrl Pts',(16.6306392094378,-18.7120365560352,-6.10552776963964));
#86269=CARTESIAN_POINT('Ctrl Pts',(16.6291723816884,-18.7251399554786,-6.10472293755726));
#86270=CARTESIAN_POINT('Ctrl Pts',(16.6282573256534,-18.7337969613771,-6.10418866430249));
#86271=CARTESIAN_POINT('Ctrl Pts',(16.6221408159027,-18.7952888771069,-6.10037676771165));
#86272=CARTESIAN_POINT('Ctrl Pts',(16.6188755558014,-18.8482929513325,-6.0970029929845));
#86273=CARTESIAN_POINT('Ctrl Pts',(16.6172125017547,-18.9177948226885,-6.09251063019151));
#86274=CARTESIAN_POINT('Ctrl Pts',(16.6170107020456,-18.9342348551601,-6.0914429592908));
#86275=CARTESIAN_POINT('Ctrl Pts',(16.6169886659508,-18.969450098497,-6.08914720684106));
#86276=CARTESIAN_POINT('Ctrl Pts',(16.6172266780594,-18.9882239675803,-6.08791797178373));
#86277=CARTESIAN_POINT('Ctrl Pts',(16.6217705576826,-19.1630888292966,-6.07643128871818));
#86278=CARTESIAN_POINT('Ctrl Pts',(16.6430861352163,-19.3182802893092,-6.06600972408595));
#86279=CARTESIAN_POINT('Ctrl Pts',(16.682457428045,-19.4743841569531,-6.05574885775411));
#86280=CARTESIAN_POINT('Ctrl Pts',(16.6836495232712,-19.4790436937119,-6.05544274146085));
#86281=CARTESIAN_POINT('Ctrl Pts',(16.7007617039586,-19.5449932002223,-6.05111238892324));
#86282=CARTESIAN_POINT('Ctrl Pts',(16.7194091640515,-19.6055472396799,-6.04716615599437));
#86283=CARTESIAN_POINT('Ctrl Pts',(16.7422893786803,-19.6694948135655,-6.0430290074528));
#86284=CARTESIAN_POINT('Ctrl Pts',(16.7438474203191,-19.6738051789005,-6.0427502863575));
#86285=CARTESIAN_POINT('Ctrl Pts',(16.745419449956,-19.6781104571528,-6.04247203196383));
#86286=CARTESIAN_POINT('Origin',(18.734,-18.952,0.));
#86287=CARTESIAN_POINT('',(16.7454193808392,-19.6781102678644,-5.2445270093495));
#86288=CARTESIAN_POINT('',(16.7454194499637,-19.6781104571739,-5.46434829365947));
#86289=CARTESIAN_POINT('',(16.7454194499637,-19.6781104571739,0.));
#86290=CARTESIAN_POINT('',(16.6170010064127,-18.9536488955056,-5.51218454189074));
#86291=CARTESIAN_POINT('Ctrl Pts',(16.7454194499637,-19.6781104571738,-5.46434829365948));
#86292=CARTESIAN_POINT('Ctrl Pts',(16.7446943071836,-19.6761245267768,-5.46447551690423));
#86293=CARTESIAN_POINT('Ctrl Pts',(16.7439721428843,-19.6741375198516,-5.46460291538803));
#86294=CARTESIAN_POINT('Ctrl Pts',(16.7420395627859,-19.668795186884,-5.46494573705574));
#86295=CARTESIAN_POINT('Ctrl Pts',(16.740834673765,-19.6654379478235,-5.46516148725336));
#86296=CARTESIAN_POINT('Ctrl Pts',(16.7382466302088,-19.6581690313182,-5.46562930939242));
#86297=CARTESIAN_POINT('Ctrl Pts',(16.7368665075815,-19.6542563823876,-5.46588155128637));
#86298=CARTESIAN_POINT('Ctrl Pts',(16.7330506743712,-19.6433362668555,-5.46658669042906));
#86299=CARTESIAN_POINT('Ctrl Pts',(16.7306403118551,-19.6363200959883,-5.46704104538664));
#86300=CARTESIAN_POINT('Ctrl Pts',(16.7169874844115,-19.5958885730821,-5.46966620983734));
#86301=CARTESIAN_POINT('Ctrl Pts',(16.7065449808684,-19.562211267477,-5.47187977553071));
#86302=CARTESIAN_POINT('Ctrl Pts',(16.6759043949841,-19.4539041773888,-5.47904995503641));
#86303=CARTESIAN_POINT('Ctrl Pts',(16.6589516976596,-19.3784249555281,-5.48412164478996));
#86304=CARTESIAN_POINT('Ctrl Pts',(16.6268475125217,-19.1870216376276,-5.49692887962248));
#86305=CARTESIAN_POINT('Ctrl Pts',(16.6170917570329,-19.0704424925791,-5.50467061913699));
#86306=CARTESIAN_POINT('Ctrl Pts',(16.6170006442156,-18.9536515473445,-5.51218500318624));
#86307=CARTESIAN_POINT('Ctrl Pts',(16.6170006421803,-18.9536489362698,-5.51218517118397));
#86308=CARTESIAN_POINT('Ctrl Pts',(16.6169350227986,-18.8694029946168,-5.51760559206411));
#86309=CARTESIAN_POINT('Ctrl Pts',(16.6218981978728,-18.7852181862553,-5.52290048669229));
#86310=CARTESIAN_POINT('Ctrl Pts',(16.6330988041816,-18.6912100105785,-5.52867287540626));
#86311=CARTESIAN_POINT('Ctrl Pts',(16.6344059040723,-18.6808876771746,-5.52930485326695));
#86312=CARTESIAN_POINT('Ctrl Pts',(16.6367383481429,-18.6634977365485,-5.53036651801471));
#86313=CARTESIAN_POINT('Ctrl Pts',(16.6377234402747,-18.6564250019566,-5.53079746726724));
#86314=CARTESIAN_POINT('Ctrl Pts',(16.6396009366482,-18.6434267198169,-5.53158795047688));
#86315=CARTESIAN_POINT('Ctrl Pts',(16.6404827461591,-18.6374997379464,-5.53194781578317));
#86316=CARTESIAN_POINT('Ctrl Pts',(16.6423536690302,-18.6252811808389,-5.53268851343968));
#86317=CARTESIAN_POINT('Ctrl Pts',(16.6433460334406,-18.618990159104,-5.53306923867726));
#86318=CARTESIAN_POINT('Ctrl Pts',(16.6456303021374,-18.6049219739914,-5.53391923499687));
#86319=CARTESIAN_POINT('Ctrl Pts',(16.6469372946277,-18.5971473298608,-5.53438802202666));
#86320=CARTESIAN_POINT('Ctrl Pts',(16.6503588000011,-18.5774675616511,-5.53557232868738));
#86321=CARTESIAN_POINT('Ctrl Pts',(16.6525319506701,-18.5655728187298,-5.53628598174709));
#86322=CARTESIAN_POINT('Ctrl Pts',(16.6655166090979,-18.4977911985791,-5.54034127620859));
#86323=CARTESIAN_POINT('Ctrl Pts',(16.6784773211522,-18.4423368536831,-5.54361371769315));
#86324=CARTESIAN_POINT('Ctrl Pts',(16.7044778550569,-18.3483651850948,-5.54912153051582));
#86325=CARTESIAN_POINT('Ctrl Pts',(16.7164193773397,-18.3095797473647,-5.55138377997392));
#86326=CARTESIAN_POINT('Ctrl Pts',(16.7772584422577,-18.1304571376729,-5.56183572081334));
#86327=CARTESIAN_POINT('Ctrl Pts',(16.8397261769852,-17.9951860173959,-5.56971124631329));
#86328=CARTESIAN_POINT('Ctrl Pts',(16.9473241089663,-17.8147856574959,-5.58140631501462));
#86329=CARTESIAN_POINT('Ctrl Pts',(16.9810917181612,-17.76339647281,-5.5848954987269));
#86330=CARTESIAN_POINT('Ctrl Pts',(17.0245031309752,-17.7032117611225,-5.58926844938547));
#86331=CARTESIAN_POINT('Ctrl Pts',(17.0320560824401,-17.6929374541602,-5.59002551701624));
#86332=CARTESIAN_POINT('Ctrl Pts',(17.0427968236048,-17.6786000334856,-5.5910978610143));
#86333=CARTESIAN_POINT('Ctrl Pts',(17.0459075357386,-17.6744791628357,-5.59140794107597));
#86334=CARTESIAN_POINT('Ctrl Pts',(17.0512483419108,-17.6674575738203,-5.59193956495328));
#86335=CARTESIAN_POINT('Ctrl Pts',(17.0534709641874,-17.6645511477927,-5.59216058428967));
#86336=CARTESIAN_POINT('Ctrl Pts',(17.057758976812,-17.6589739248193,-5.59258659438384));
#86337=CARTESIAN_POINT('Ctrl Pts',(17.0598232317183,-17.6563022933221,-5.59279150036745));
#86338=CARTESIAN_POINT('Ctrl Pts',(17.0653350907805,-17.6492038133727,-5.59333813627106));
#86339=CARTESIAN_POINT('Ctrl Pts',(17.0687938905799,-17.6447857502881,-5.59368065136171));
#86340=CARTESIAN_POINT('Ctrl Pts',(17.08127082961,-17.6289783317728,-5.59491422656436));
#86341=CARTESIAN_POINT('Ctrl Pts',(17.0903883505925,-17.6176684202998,-5.59581197951903));
#86342=CARTESIAN_POINT('Ctrl Pts',(17.200503309865,-17.4839164000592,-5.60660193792685));
#86343=CARTESIAN_POINT('Ctrl Pts',(17.3148381850228,-17.3731221783315,-5.61724586839603));
#86344=CARTESIAN_POINT('Ctrl Pts',(17.5176005004806,-17.2166167868411,-5.63410078951487));
#86345=CARTESIAN_POINT('Ctrl Pts',(17.5987568061117,-17.1624723268067,-5.64042665492986));
#86346=CARTESIAN_POINT('Ctrl Pts',(17.7122850875287,-17.0975735432327,-5.64865929151614));
#86347=CARTESIAN_POINT('Ctrl Pts',(17.7415946565475,-17.0817244391084,-5.65073406370446));
#86348=CARTESIAN_POINT('Ctrl Pts',(17.7854570821705,-17.0593275041427,-5.65376557909403));
#86349=CARTESIAN_POINT('Ctrl Pts',(17.7997283748285,-17.0522422797378,-5.65474072790219));
#86350=CARTESIAN_POINT('Ctrl Pts',(17.8257475257002,-17.0396887536952,-5.65649867414142));
#86351=CARTESIAN_POINT('Ctrl Pts',(17.8374680790026,-17.0341659649094,-5.65728333088977));
#86352=CARTESIAN_POINT('Ctrl Pts',(17.8559004135295,-17.0256864520797,-5.65850623506506));
#86353=CARTESIAN_POINT('Ctrl Pts',(17.8625779659465,-17.0226564822884,-5.65894700383009));
#86354=CARTESIAN_POINT('Ctrl Pts',(17.8693096748947,-17.0196440174112,-5.65938910762456));
#86355=CARTESIAN_POINT('Ctrl Pts',(17.8693481578123,-17.0196267975417,-5.65939163490994));
#86356=CARTESIAN_POINT('Ctrl Pts',(17.8694264533099,-17.0195917656287,-5.65939677665411));
#86357=CARTESIAN_POINT('Ctrl Pts',(17.8694662658332,-17.0195739537075,-5.65939939110402));
#86358=CARTESIAN_POINT('Ctrl Pts',(17.8695472699262,-17.0195377158909,-5.65940471040463));
#86359=CARTESIAN_POINT('Ctrl Pts',(17.8695884614128,-17.0195192901368,-5.65940741524432));
#86360=CARTESIAN_POINT('Ctrl Pts',(17.8696722746066,-17.0194818020789,-5.65941291866806));
#86361=CARTESIAN_POINT('Ctrl Pts',(17.8697148964165,-17.0194627398408,-5.65941571725291));
#86362=CARTESIAN_POINT('Ctrl Pts',(17.8698016326997,-17.0194239512271,-5.65942141224898));
#86363=CARTESIAN_POINT('Ctrl Pts',(17.8698457336059,-17.0194042310392,-5.6594243077628));
#86364=CARTESIAN_POINT('Ctrl Pts',(17.8699354782875,-17.0193641044377,-5.65943019989428));
#86365=CARTESIAN_POINT('Ctrl Pts',(17.8699811233137,-17.0193436975943,-5.65943319658701));
#86366=CARTESIAN_POINT('Ctrl Pts',(17.8700740092451,-17.0193021743753,-5.65943929453521));
#86367=CARTESIAN_POINT('Ctrl Pts',(17.8701212512532,-17.0192810576444,-5.6594423958558));
#86368=CARTESIAN_POINT('Ctrl Pts',(17.8702173914648,-17.0192380881082,-5.6594487069971));
#86369=CARTESIAN_POINT('Ctrl Pts',(17.8702662906793,-17.0192162349992,-5.65945191687633));
#86370=CARTESIAN_POINT('Ctrl Pts',(17.8703658080825,-17.0191717651008,-5.65945844923198));
#86371=CARTESIAN_POINT('Ctrl Pts',(17.8704164271829,-17.0191491480631,-5.65946177175981));
#86372=CARTESIAN_POINT('Ctrl Pts',(17.8705194496144,-17.0191031216335,-5.65946853367027));
#86373=CARTESIAN_POINT('Ctrl Pts',(17.8705718539176,-17.0190797119783,-5.65947197310764));
#86374=CARTESIAN_POINT('Ctrl Pts',(17.8706785147643,-17.0190320704522,-5.65947897327325));
#86375=CARTESIAN_POINT('Ctrl Pts',(17.8707327721683,-17.0190078383806,-5.65948253404822));
#86376=CARTESIAN_POINT('Ctrl Pts',(17.8708432101602,-17.0189585208956,-5.65948978151524));
#86377=CARTESIAN_POINT('Ctrl Pts',(17.8708993913897,-17.018933435393,-5.65949346823892));
#86378=CARTESIAN_POINT('Ctrl Pts',(17.8710137506744,-17.0188823787639,-5.659500972404));
#86379=CARTESIAN_POINT('Ctrl Pts',(17.8710719295412,-17.0188564074873,-5.65950478988741));
#86380=CARTESIAN_POINT('Ctrl Pts',(17.8711903608708,-17.0188035456843,-5.6595125605751));
#86381=CARTESIAN_POINT('Ctrl Pts',(17.8712506139923,-17.0187766550922,-5.65951651381048));
#86382=CARTESIAN_POINT('Ctrl Pts',(17.8713732738242,-17.0187219196513,-5.65952456121369));
#86383=CARTESIAN_POINT('Ctrl Pts',(17.8714356811169,-17.0186940747881,-5.65952865540668));
#86384=CARTESIAN_POINT('Ctrl Pts',(17.8715627324487,-17.0186373944475,-5.65953699014101));
#86385=CARTESIAN_POINT('Ctrl Pts',(17.871627377147,-17.0186085589401,-5.65954123071157));
#86386=CARTESIAN_POINT('Ctrl Pts',(17.8717589900414,-17.0185498594166,-5.65954986384918));
#86387=CARTESIAN_POINT('Ctrl Pts',(17.8718259586386,-17.0185199955058,-5.65955425642745));
#86388=CARTESIAN_POINT('Ctrl Pts',(17.8719623113204,-17.0184591990169,-5.65956319956844));
#86389=CARTESIAN_POINT('Ctrl Pts',(17.8720316931899,-17.0184282677323,-5.65956774996957));
#86390=CARTESIAN_POINT('Ctrl Pts',(17.8721597313376,-17.0183711950234,-5.65957614689648));
#86391=CARTESIAN_POINT('Ctrl Pts',(17.8722183884455,-17.0183450519521,-5.65957999354451));
#86392=CARTESIAN_POINT('Ctrl Pts',(17.8723455735027,-17.0182883733799,-5.65958833378747));
#86393=CARTESIAN_POINT('Ctrl Pts',(17.8724141029666,-17.018257838371,-5.65959282741978));
#86394=CARTESIAN_POINT('Ctrl Pts',(17.8725627043293,-17.0181916348017,-5.65960257104508));
#86395=CARTESIAN_POINT('Ctrl Pts',(17.8726427776966,-17.018155967181,-5.65960782104974));
#86396=CARTESIAN_POINT('Ctrl Pts',(17.8728164233179,-17.0180786319644,-5.65961920542613));
#86397=CARTESIAN_POINT('Ctrl Pts',(17.8729099970741,-17.0180369658773,-5.65962533978073));
#86398=CARTESIAN_POINT('Ctrl Pts',(17.8731129330203,-17.0179466211511,-5.65963864258498));
#86399=CARTESIAN_POINT('Ctrl Pts',(17.8732222968437,-17.0178979447612,-5.65964581098369));
#86400=CARTESIAN_POINT('Ctrl Pts',(17.8734594918218,-17.01779239652,-5.65966135696751));
#86401=CARTESIAN_POINT('Ctrl Pts',(17.8735873239917,-17.0177355282849,-5.65966973440319));
#86402=CARTESIAN_POINT('Ctrl Pts',(17.8738603533401,-17.0176140991275,-5.65968762556345));
#86403=CARTESIAN_POINT('Ctrl Pts',(17.8740055521962,-17.0175495418603,-5.65969713916434));
#86404=CARTESIAN_POINT('Ctrl Pts',(17.8800513360354,-17.0148623243139,-5.66009322281979));
#86405=CARTESIAN_POINT('Ctrl Pts',(17.8859639318968,-17.0122666358823,-5.66047886515401));
#86406=CARTESIAN_POINT('Ctrl Pts',(17.8996478086091,-17.0063338036385,-5.66136747146807));
#86407=CARTESIAN_POINT('Ctrl Pts',(17.9074274292356,-17.0030160812955,-5.66186976848795));
#86408=CARTESIAN_POINT('Ctrl Pts',(17.928413223001,-16.994214666736,-5.66321708880192));
#86409=CARTESIAN_POINT('Ctrl Pts',(17.9416555621867,-16.988817946999,-5.66405916577417));
#86410=CARTESIAN_POINT('Ctrl Pts',(18.0634385186055,-16.9406200923856,-5.67173194859101));
#86411=CARTESIAN_POINT('Ctrl Pts',(18.1752954471009,-16.906723416681,-5.6782469384445));
#86412=CARTESIAN_POINT('Ctrl Pts',(18.4481258427835,-16.8481167008556,-5.69352434138673));
#86413=CARTESIAN_POINT('Ctrl Pts',(18.6102383492975,-16.8323961832075,-5.70210470895674));
#86414=CARTESIAN_POINT('Ctrl Pts',(18.8054972418901,-16.8359508169542,-5.71331233068431));
#86415=CARTESIAN_POINT('Ctrl Pts',(18.8384409162346,-16.8373208697635,-5.71523458434318));
#86416=CARTESIAN_POINT('Ctrl Pts',(18.8785926222888,-16.8399311470804,-5.71763013311381));
#86417=CARTESIAN_POINT('Ctrl Pts',(18.8858456019452,-16.8404402031728,-5.71806496797585));
#86418=CARTESIAN_POINT('Ctrl Pts',(18.8972006262636,-16.8412959701197,-5.7187492280128));
#86419=CARTESIAN_POINT('Ctrl Pts',(18.9013046059562,-16.8416173061911,-5.71899725215569));
#86420=CARTESIAN_POINT('Ctrl Pts',(18.9089668395643,-16.8422397394575,-5.71946170027918));
#86421=CARTESIAN_POINT('Ctrl Pts',(18.9125252777922,-16.8425378703443,-5.71967795634331));
#86422=CARTESIAN_POINT('Ctrl Pts',(18.9206372324492,-16.8432381737941,-5.72017221190029));
#86423=CARTESIAN_POINT('Ctrl Pts',(18.9251901942608,-16.843646091162,-5.72045052974823));
#86424=CARTESIAN_POINT('Ctrl Pts',(18.93704612942,-16.844747029102,-5.721177576326));
#86425=CARTESIAN_POINT('Ctrl Pts',(18.944346813191,-16.8454632619812,-5.72162755942545));
#86426=CARTESIAN_POINT('Ctrl Pts',(18.9915467508741,-16.8503416192697,-5.7245508748871));
#86427=CARTESIAN_POINT('Ctrl Pts',(19.0313218380476,-16.8555989115244,-5.72707950848353));
#86428=CARTESIAN_POINT('Ctrl Pts',(19.2554634123781,-16.8917315644293,-5.74161077908658));
#86429=CARTESIAN_POINT('Ctrl Pts',(19.4352570585357,-16.9457900248012,-5.75426243444807));
#86430=CARTESIAN_POINT('Ctrl Pts',(19.6769844769193,-17.0550022500074,-5.77133966825835));
#86431=CARTESIAN_POINT('Ctrl Pts',(19.7465040706997,-17.0911781063814,-5.77627398346786));
#86432=CARTESIAN_POINT('Ctrl Pts',(19.8304196120095,-17.140944115937,-5.7822535054873));
#86433=CARTESIAN_POINT('Ctrl Pts',(19.8468386260565,-17.15098650434,-5.7834248383092));
#86434=CARTESIAN_POINT('Ctrl Pts',(19.8704224628136,-17.1658567985635,-5.78510977979849));
#86435=CARTESIAN_POINT('Ctrl Pts',(19.8776979144243,-17.1705066281298,-5.78562992083963));
#86436=CARTESIAN_POINT('Ctrl Pts',(19.89036817752,-17.1787139563357,-5.78653643052581));
#86437=CARTESIAN_POINT('Ctrl Pts',(19.8957754877898,-17.1822518619751,-5.7869235218915));
#86438=CARTESIAN_POINT('Ctrl Pts',(19.9062179450938,-17.1891526586306,-5.78767152365043));
#86439=CARTESIAN_POINT('Ctrl Pts',(19.9112550242194,-17.192512498227,-5.78803254332648));
#86440=CARTESIAN_POINT('Ctrl Pts',(19.9232211596349,-17.2005685574896,-5.78889072630208));
#86441=CARTESIAN_POINT('Ctrl Pts',(19.9301369475409,-17.2052843762867,-5.78938714531626));
#86442=CARTESIAN_POINT('Ctrl Pts',(19.9547609130254,-17.2222900808458,-5.79115640509348));
#86443=CARTESIAN_POINT('Ctrl Pts',(19.9723095139871,-17.234809501203,-5.79242051212765));
#86444=CARTESIAN_POINT('Ctrl Pts',(20.1431267712248,-17.3606535062871,-5.80476723875693));
#86445=CARTESIAN_POINT('Ctrl Pts',(20.2806128910576,-17.4939135859242,-5.81493699732937));
#86446=CARTESIAN_POINT('Ctrl Pts',(20.4459354991579,-17.7042499463965,-5.829537841401));
#86447=CARTESIAN_POINT('Ctrl Pts',(20.490125763983,-17.7672536903842,-5.83377648366255));
#86448=CARTESIAN_POINT('Ctrl Pts',(20.5493717944037,-17.8623443803206,-5.84019112560869));
#86449=CARTESIAN_POINT('Ctrl Pts',(20.5672094732885,-17.8926290435782,-5.84223672412439));
#86450=CARTESIAN_POINT('Ctrl Pts',(20.5878853854289,-17.9298195305303,-5.84476930748475));
#86451=CARTESIAN_POINT('Ctrl Pts',(20.5914526923786,-17.936316276413,-5.84521246473651));
#86452=CARTESIAN_POINT('Ctrl Pts',(20.5969628220267,-17.9464773871417,-5.84590694501551));
#86453=CARTESIAN_POINT('Ctrl Pts',(20.5989291562691,-17.950129028945,-5.84615679739511));
#86454=CARTESIAN_POINT('Ctrl Pts',(20.6025667278976,-17.956932108814,-5.84662283028362));
#86455=CARTESIAN_POINT('Ctrl Pts',(20.6042407351354,-17.9600820010215,-5.84683883153487));
#86456=CARTESIAN_POINT('Ctrl Pts',(20.6080210937815,-17.9672388955982,-5.84733010967557));
#86457=CARTESIAN_POINT('Ctrl Pts',(20.6101225486658,-17.9712484136192,-5.84760568970901));
#86458=CARTESIAN_POINT('Ctrl Pts',(20.616328450418,-17.983182038179,-5.84842687485972));
#86459=CARTESIAN_POINT('Ctrl Pts',(20.6203956094586,-17.9911252752903,-5.84897473663431));
#86460=CARTESIAN_POINT('Ctrl Pts',(20.650873827475,-18.0515891501038,-5.85315327381671));
#86461=CARTESIAN_POINT('Ctrl Pts',(20.6751347407946,-18.1051590765481,-5.85690168862045));
#86462=CARTESIAN_POINT('Ctrl Pts',(20.7573841374128,-18.3089442862489,-5.87115228501349));
#86463=CARTESIAN_POINT('Ctrl Pts',(20.8004134778637,-18.4646133598965,-5.88197243785938));
#86464=CARTESIAN_POINT('Ctrl Pts',(20.83827332445,-18.7057689371455,-5.89773293319788));
#86465=CARTESIAN_POINT('Ctrl Pts',(20.8463182405322,-18.7885665658537,-5.90298236303472));
#86466=CARTESIAN_POINT('Ctrl Pts',(20.8502283583189,-18.891490113137,-5.90929917240716));
#86467=CARTESIAN_POINT('Ctrl Pts',(20.850703145337,-18.911358300341,-5.91050920873632));
#86468=CARTESIAN_POINT('Ctrl Pts',(20.8509839287434,-18.9399770784174,-5.91223922545566));
#86469=CARTESIAN_POINT('Ctrl Pts',(20.8510155351723,-18.948723930948,-5.91276623586004));
#86470=CARTESIAN_POINT('Ctrl Pts',(20.8509761845312,-18.9639510534059,-5.91368073249653));
#86471=CARTESIAN_POINT('Ctrl Pts',(20.8509296835682,-18.9704312187982,-5.91406897946326));
#86472=CARTESIAN_POINT('Ctrl Pts',(20.8507825313564,-18.9829356586667,-5.9148163954341));
#86473=CARTESIAN_POINT('Ctrl Pts',(20.8506859158304,-18.9889599095375,-5.91517568702399));
#86474=CARTESIAN_POINT('Ctrl Pts',(20.8503959608,-19.0032376021382,-5.91602538732019));
#86475=CARTESIAN_POINT('Ctrl Pts',(20.8501800573199,-19.0114905261439,-5.9165150860796));
#86476=CARTESIAN_POINT('Ctrl Pts',(20.8492481751235,-19.0405977626733,-5.91823724521997));
#86477=CARTESIAN_POINT('Ctrl Pts',(20.8482721414848,-19.0614429690031,-5.9194615755354));
#86478=CARTESIAN_POINT('Ctrl Pts',(20.8349195301613,-19.2780217101206,-5.93209802108429));
#86479=CARTESIAN_POINT('Ctrl Pts',(20.7957116125451,-19.471136842044,-5.94253264527725));
#86480=CARTESIAN_POINT('Ctrl Pts',(20.7060363475559,-19.725409376425,-5.95726787856034));
#86481=CARTESIAN_POINT('Ctrl Pts',(20.6780044229229,-19.7933884761063,-5.96132793154709));
#86482=CARTESIAN_POINT('Ctrl Pts',(20.6318415645186,-19.890645122005,-5.96749811587761));
#86483=CARTESIAN_POINT('Ctrl Pts',(20.6164405123277,-19.9211618470911,-5.96948906163561));
#86484=CARTESIAN_POINT('Ctrl Pts',(20.5968388670197,-19.9577705438264,-5.97196095558192));
#86485=CARTESIAN_POINT('Ctrl Pts',(20.5933354846469,-19.9642324748997,-5.97240049907114));
#86486=CARTESIAN_POINT('Ctrl Pts',(20.5878093207955,-19.9742999034154,-5.97309054237961));
#86487=CARTESIAN_POINT('Ctrl Pts',(20.5858094709634,-19.9779180147411,-5.97333960195996));
#86488=CARTESIAN_POINT('Ctrl Pts',(20.5820635311024,-19.9846484981735,-5.97380494150045));
#86489=CARTESIAN_POINT('Ctrl Pts',(20.580320164469,-19.9877623209086,-5.97402104710093));
#86490=CARTESIAN_POINT('Ctrl Pts',(20.5763382018878,-19.994832495569,-5.97451358841931));
#86491=CARTESIAN_POINT('Ctrl Pts',(20.574094740651,-19.9987860375872,-5.97479033376068));
#86492=CARTESIAN_POINT('Ctrl Pts',(20.5682393351684,-20.009027742675,-5.97551062455493));
#86493=CARTESIAN_POINT('Ctrl Pts',(20.5646078179868,-20.0153045663024,-5.97595538722397));
#86494=CARTESIAN_POINT('Ctrl Pts',(20.5414281557698,-20.0548982776846,-5.97878136511788));
#86495=CARTESIAN_POINT('Ctrl Pts',(20.5210047429295,-20.0876913164861,-5.98121385426217));
#86496=CARTESIAN_POINT('Ctrl Pts',(20.4925758994939,-20.1306714727416,-5.98450801605362));
#86497=CARTESIAN_POINT('Ctrl Pts',(20.4853562319744,-20.1413725115899,-5.98533723008799));
#86498=CARTESIAN_POINT('Ctrl Pts',(20.4775930864207,-20.1526551414211,-5.98622064873828));
#86499=CARTESIAN_POINT('Ctrl Pts',(20.4771465239886,-20.1533033819726,-5.98627143756127));
#86500=CARTESIAN_POINT('Ctrl Pts',(20.4637351643345,-20.1727484041632,-5.98779589475466));
#86501=CARTESIAN_POINT('Ctrl Pts',(20.4504677719701,-20.1913339906392,-5.98928001143226));
#86502=CARTESIAN_POINT('Ctrl Pts',(20.4097690239052,-20.2464393109292,-5.99375473987897));
#86503=CARTESIAN_POINT('Ctrl Pts',(20.3814541667607,-20.2822892651614,-5.99676602233453));
#86504=CARTESIAN_POINT('Ctrl Pts',(20.2814846202797,-20.400771285459,-6.00700642808005));
#86505=CARTESIAN_POINT('Ctrl Pts',(20.2045912823814,-20.478765088136,-6.01423700915862));
#86506=CARTESIAN_POINT('Ctrl Pts',(20.0804340602093,-20.5865753048392,-6.02480599869715));
#86507=CARTESIAN_POINT('Ctrl Pts',(20.0374614715426,-20.6210446720852,-6.02829279981356));
#86508=CARTESIAN_POINT('Ctrl Pts',(19.9656280358225,-20.674195396578,-6.03384708465625));
#86509=CARTESIAN_POINT('Ctrl Pts',(19.9375730022023,-20.6939175775582,-6.0359529505016));
#86510=CARTESIAN_POINT('Ctrl Pts',(19.900060847423,-20.7189487492393,-6.03868839018908));
#86511=CARTESIAN_POINT('Ctrl Pts',(19.8910258513193,-20.7248781595169,-6.03934128212492));
#86512=CARTESIAN_POINT('Ctrl Pts',(19.876150233645,-20.734478448887,-6.04040664527257));
#86513=CARTESIAN_POINT('Ctrl Pts',(19.8703364545421,-20.738190370815,-6.04082064517096));
#86514=CARTESIAN_POINT('Ctrl Pts',(19.8590454245858,-20.7453219131538,-6.04162014506751));
#86515=CARTESIAN_POINT('Ctrl Pts',(19.8535704732395,-20.7487450148686,-6.04200577123864));
#86516=CARTESIAN_POINT('Ctrl Pts',(19.840889846732,-20.7565928529328,-6.04289425940899));
#86517=CARTESIAN_POINT('Ctrl Pts',(19.8336731210191,-20.7609995930699,-6.04339645501683));
#86518=CARTESIAN_POINT('Ctrl Pts',(19.8141869501236,-20.7727387095206,-6.04474332372036));
#86519=CARTESIAN_POINT('Ctrl Pts',(19.8018691957539,-20.7799903422187,-6.04558505361947));
#86520=CARTESIAN_POINT('Ctrl Pts',(19.687971721121,-20.8454991751386,-6.05328244033555));
#86521=CARTESIAN_POINT('Ctrl Pts',(19.5817897889601,-20.895362789935,-6.05981987563774));
#86522=CARTESIAN_POINT('Ctrl Pts',(19.3186488225908,-20.9932374225985,-6.07518824952006));
#86523=CARTESIAN_POINT('Ctrl Pts',(19.1592049096371,-21.0323011801609,-6.08383349797618));
#86524=CARTESIAN_POINT('Ctrl Pts',(18.9656474453625,-21.0565234569939,-6.09504685944817));
#86525=CARTESIAN_POINT('Ctrl Pts',(18.9343370969792,-21.0597344066654,-6.09688397808098));
#86526=CARTESIAN_POINT('Ctrl Pts',(18.8958241196297,-21.0628181654,-6.09918478879517));
#86527=CARTESIAN_POINT('Ctrl Pts',(18.888676741851,-21.0633539436256,-6.09961351470817));
#86528=CARTESIAN_POINT('Ctrl Pts',(18.8774430253808,-21.064138692859,-6.1002902684027));
#86529=CARTESIAN_POINT('Ctrl Pts',(18.8733583737348,-21.0644121289226,-6.10053694532106));
#86530=CARTESIAN_POINT('Ctrl Pts',(18.8657059619658,-21.064902107403,-6.10100025901778));
#86531=CARTESIAN_POINT('Ctrl Pts',(18.8621384378512,-21.0651214626611,-6.10121673634778));
#86532=CARTESIAN_POINT('Ctrl Pts',(18.853972511504,-21.0656028033679,-6.10171333840958));
#86533=CARTESIAN_POINT('Ctrl Pts',(18.8493738127962,-21.0658588165524,-6.10199379334528));
#86534=CARTESIAN_POINT('Ctrl Pts',(18.8351628233966,-21.0666034423847,-6.10286282430619));
#86535=CARTESIAN_POINT('Ctrl Pts',(18.8255481651871,-21.0670415033285,-6.10345412012196));
#86536=CARTESIAN_POINT('Ctrl Pts',(18.7294012836835,-21.0707653212148,-6.10939822993797));
#86537=CARTESIAN_POINT('Ctrl Pts',(18.6427568672297,-21.0688039239774,-6.11500403451157));
#86538=CARTESIAN_POINT('Ctrl Pts',(18.4300122787677,-21.0509020042212,-6.12902167268099));
#86539=CARTESIAN_POINT('Ctrl Pts',(18.304740786168,-21.028905934046,-6.13748305759993));
#86540=CARTESIAN_POINT('Ctrl Pts',(18.0889892583227,-20.9706555573753,-6.15194729410804));
#86541=CARTESIAN_POINT('Ctrl Pts',(17.9976065088923,-20.9391432458174,-6.15804197531535));
#86542=CARTESIAN_POINT('Ctrl Pts',(17.8952172254498,-20.8957968701017,-6.16482090748904));
#86543=CARTESIAN_POINT('Ctrl Pts',(17.8818109387683,-20.8899568199136,-6.16570766687662));
#86544=CARTESIAN_POINT('Ctrl Pts',(17.8614116580938,-20.8808178599124,-6.16705593554101));
#86545=CARTESIAN_POINT('Ctrl Pts',(17.8543746394194,-20.8776188560157,-6.16752084917421));
#86546=CARTESIAN_POINT('Ctrl Pts',(17.8415803463361,-20.8717178452156,-6.16836583266904));
#86547=CARTESIAN_POINT('Ctrl Pts',(17.8358174493384,-20.8690283123987,-6.16874632639375));
#86548=CARTESIAN_POINT('Ctrl Pts',(17.8233758156527,-20.8631534069505,-6.16956758342424));
#86549=CARTESIAN_POINT('Ctrl Pts',(17.8167014673545,-20.8599588973965,-6.17000802446731));
#86550=CARTESIAN_POINT('Ctrl Pts',(17.7985847189788,-20.8511707308412,-6.17120329790977));
#86551=CARTESIAN_POINT('Ctrl Pts',(17.7871757127367,-20.8455086460224,-6.17195574260547));
#86552=CARTESIAN_POINT('Ctrl Pts',(17.7311353646994,-20.8170636663194,-6.17565124543442));
#86553=CARTESIAN_POINT('Ctrl Pts',(17.6872694976211,-20.7928030293878,-6.17854193722928));
#86554=CARTESIAN_POINT('Ctrl Pts',(17.4954798087589,-20.6776560301375,-6.19124130415125));
#86555=CARTESIAN_POINT('Ctrl Pts',(17.3582178045451,-20.5703461393829,-6.20043478884896));
#86556=CARTESIAN_POINT('Ctrl Pts',(17.1912971766094,-20.4030992892138,-6.21342103395186));
#86557=CARTESIAN_POINT('Ctrl Pts',(17.1489970438489,-20.3567724473044,-6.21691352420763));
#86558=CARTESIAN_POINT('Ctrl Pts',(17.0889997131088,-20.2848989097309,-6.22229878014459));
#86559=CARTESIAN_POINT('Ctrl Pts',(17.0697048391059,-20.2607271823504,-6.22410480465985));
#86560=CARTESIAN_POINT('Ctrl Pts',(17.046623499201,-20.2304757950802,-6.2263709770117));
#86561=CARTESIAN_POINT('Ctrl Pts',(17.0423282330767,-20.22478688073,-6.22679739217315));
#86562=CARTESIAN_POINT('Ctrl Pts',(17.0356167565575,-20.215803800939,-6.22747130569117));
#86563=CARTESIAN_POINT('Ctrl Pts',(17.0331811648282,-20.2125240886831,-6.22771747195634));
#86564=CARTESIAN_POINT('Ctrl Pts',(17.0286315569084,-20.2063604981061,-6.22818036358819));
#86565=CARTESIAN_POINT('Ctrl Pts',(17.0265153489955,-20.2034783065662,-6.2283969327432));
#86566=CARTESIAN_POINT('Ctrl Pts',(17.021681949478,-20.1968603267421,-6.22889446050305));
#86567=CARTESIAN_POINT('Ctrl Pts',(17.0189696845702,-20.1931210075826,-6.22917575395577));
#86568=CARTESIAN_POINT('Ctrl Pts',(17.0106032965739,-20.1815067251903,-6.23004992143128));
#86569=CARTESIAN_POINT('Ctrl Pts',(17.0049911062667,-20.1736019080929,-6.23064556095518));
#86570=CARTESIAN_POINT('Ctrl Pts',(16.9421416851821,-20.0837772550423,-6.23741893712719));
#86571=CARTESIAN_POINT('Ctrl Pts',(16.8907261923401,-19.9979507172628,-6.24393186162075));
#86572=CARTESIAN_POINT('Ctrl Pts',(16.8076114278052,-19.8339121607158,-6.25604812770089));
#86573=CARTESIAN_POINT('Ctrl Pts',(16.7741769643098,-19.7568679012229,-6.26161628492563));
#86574=CARTESIAN_POINT('Ctrl Pts',(16.7454195726558,-19.6781107931876,-6.26710635146282));
#86575=CARTESIAN_POINT('',(16.617000284924,-18.950901652078,-5.287306223149));
#86576=CARTESIAN_POINT('Ctrl Pts',(16.745419449956,-19.6781104571528,-6.04247203196383));
#86577=CARTESIAN_POINT('Ctrl Pts',(16.7481387492912,-19.6855577342365,-6.04199070707657));
#86578=CARTESIAN_POINT('Ctrl Pts',(16.7508999037001,-19.6929897896995,-6.04151077890519));
#86579=CARTESIAN_POINT('Ctrl Pts',(16.7565355594176,-19.7079018417615,-6.04054860527923));
#86580=CARTESIAN_POINT('Ctrl Pts',(16.7594108953478,-19.7153813455215,-6.04006639995054));
#86581=CARTESIAN_POINT('Ctrl Pts',(16.7646516739141,-19.7287862461309,-6.03920283878544));
#86582=CARTESIAN_POINT('Ctrl Pts',(16.7670015547204,-19.734717585904,-6.03882096602459));
#86583=CARTESIAN_POINT('Ctrl Pts',(16.7720578574421,-19.7473136300662,-6.03801046018694));
#86584=CARTESIAN_POINT('Ctrl Pts',(16.7747715122763,-19.7539753585776,-6.03758207679116));
#86585=CARTESIAN_POINT('Ctrl Pts',(16.7821570623799,-19.771844853206,-6.03643363270401));
#86586=CARTESIAN_POINT('Ctrl Pts',(16.7868915607623,-19.783026576937,-6.0357156995046));
#86587=CARTESIAN_POINT('Ctrl Pts',(16.8108500261443,-19.8382816408423,-6.03217068491787));
#86588=CARTESIAN_POINT('Ctrl Pts',(16.831476300288,-19.881733865292,-6.02939189453329));
#86589=CARTESIAN_POINT('Ctrl Pts',(16.930577056764,-20.0733660666286,-6.01711721964233));
#86590=CARTESIAN_POINT('Ctrl Pts',(17.0250013165618,-20.2126035042643,-6.00819923758914));
#86591=CARTESIAN_POINT('Ctrl Pts',(17.199551880873,-20.4138148562186,-5.99361572160997));
#86592=CARTESIAN_POINT('Ctrl Pts',(17.2693672499324,-20.4837569939524,-5.98812307736492));
#86593=CARTESIAN_POINT('Ctrl Pts',(17.3511068479787,-20.5549315408755,-5.98170194278436));
#86594=CARTESIAN_POINT('Ctrl Pts',(17.3584620216197,-20.5612477300285,-5.98112420455132));
#86595=CARTESIAN_POINT('Ctrl Pts',(17.3693853990106,-20.5704984803597,-5.98026582182577));
#86596=CARTESIAN_POINT('Ctrl Pts',(17.3729203611795,-20.5734723420463,-5.97998798066685));
#86597=CARTESIAN_POINT('Ctrl Pts',(17.3792087466741,-20.5787275265782,-5.97949356826934));
#86598=CARTESIAN_POINT('Ctrl Pts',(17.3819582460412,-20.5810134686855,-5.97927733901209));
#86599=CARTESIAN_POINT('Ctrl Pts',(17.3878614400673,-20.5858961612704,-5.97881295821649));
#86600=CARTESIAN_POINT('Ctrl Pts',(17.3910168158417,-20.5884907133155,-5.97856466042602));
#86601=CARTESIAN_POINT('Ctrl Pts',(17.3996985525994,-20.595587374442,-5.97788132804067));
#86602=CARTESIAN_POINT('Ctrl Pts',(17.4052401142143,-20.600070681905,-5.9774449759169));
#86603=CARTESIAN_POINT('Ctrl Pts',(17.4349421974628,-20.6238534713412,-5.9751057122744));
#86604=CARTESIAN_POINT('Ctrl Pts',(17.4594994153522,-20.6426487602319,-5.97317002821319));
#86605=CARTESIAN_POINT('Ctrl Pts',(17.5350662192519,-20.6979030162766,-5.96723065921933));
#86606=CARTESIAN_POINT('Ctrl Pts',(17.587290050673,-20.7326388590416,-5.96314954411795));
#86607=CARTESIAN_POINT('Ctrl Pts',(17.7561737857018,-20.834455697973,-5.95019052642287));
#86608=CARTESIAN_POINT('Ctrl Pts',(17.8777423218272,-20.8927760163412,-5.9412248743718));
#86609=CARTESIAN_POINT('Ctrl Pts',(18.0423575389777,-20.9532464173255,-5.92993142488277));
#86610=CARTESIAN_POINT('Ctrl Pts',(18.0810894524547,-20.9662156421424,-5.92732947852865));
#86611=CARTESIAN_POINT('Ctrl Pts',(18.1665837467932,-20.9921174813466,-5.92171050148367));
#86612=CARTESIAN_POINT('Ctrl Pts',(18.213465361283,-21.0045800438516,-5.91870888879738));
#86613=CARTESIAN_POINT('Ctrl Pts',(18.2730119749151,-21.0182375578628,-5.91499301897416));
#86614=CARTESIAN_POINT('Ctrl Pts',(18.2853121651644,-21.0209434120858,-5.91423055066757));
#86615=CARTESIAN_POINT('Ctrl Pts',(18.3048443021115,-21.0250578024833,-5.91302768013504));
#86616=CARTESIAN_POINT('Ctrl Pts',(18.3120605690662,-21.0265385955021,-5.91258497251876));
#86617=CARTESIAN_POINT('Ctrl Pts',(18.3255226958963,-21.0292279028188,-5.9117622075774));
#86618=CARTESIAN_POINT('Ctrl Pts',(18.3317665390026,-21.0304459849698,-5.91138184856124));
#86619=CARTESIAN_POINT('Ctrl Pts',(18.3456487633709,-21.0330893039478,-5.91053890314906));
#86620=CARTESIAN_POINT('Ctrl Pts',(18.3532897159894,-21.0345006737356,-5.91007676338969));
#86621=CARTESIAN_POINT('Ctrl Pts',(18.3755207657643,-21.0384805536681,-5.90873738525707));
#86622=CARTESIAN_POINT('Ctrl Pts',(18.3901304551278,-21.0409380591613,-5.9078636782931));
#86623=CARTESIAN_POINT('Ctrl Pts',(18.506761463762,-21.0592998779833,-5.90093807131005));
#86624=CARTESIAN_POINT('Ctrl Pts',(18.6098026865321,-21.067875510353,-5.89512919743182));
#86625=CARTESIAN_POINT('Ctrl Pts',(18.872705181404,-21.0704748771832,-5.88065401722067));
#86626=CARTESIAN_POINT('Ctrl Pts',(19.0319912381937,-21.0539914986133,-5.87222578509501));
#86627=CARTESIAN_POINT('Ctrl Pts',(19.235308715798,-21.0093610985793,-5.86047071994354));
#86628=CARTESIAN_POINT('Ctrl Pts',(19.2823439196685,-20.9973271806295,-5.85767580525113));
#86629=CARTESIAN_POINT('Ctrl Pts',(19.3363657926869,-20.9815084741173,-5.85433393032942));
#86630=CARTESIAN_POINT('Ctrl Pts',(19.3437994923213,-20.9792872933324,-5.85387113548219));
#86631=CARTESIAN_POINT('Ctrl Pts',(19.3556664429391,-20.9756702880281,-5.85312739398144));
#86632=CARTESIAN_POINT('Ctrl Pts',(19.3601076775438,-20.9743006146719,-5.85284793443878));
#86633=CARTESIAN_POINT('Ctrl Pts',(19.3679697913483,-20.9718475635104,-5.85235118750972));
#86634=CARTESIAN_POINT('Ctrl Pts',(19.3713924687732,-20.9707701000234,-5.85213424864671));
#86635=CARTESIAN_POINT('Ctrl Pts',(19.3786459916911,-20.9684663954237,-5.85167302286242));
#86636=CARTESIAN_POINT('Ctrl Pts',(19.3824760267831,-20.9672379563071,-5.85142861365488));
#86637=CARTESIAN_POINT('Ctrl Pts',(19.3928136955816,-20.9638897478543,-5.85076661739924));
#86638=CARTESIAN_POINT('Ctrl Pts',(19.3993145230052,-20.961749343955,-5.85034784399367));
#86639=CARTESIAN_POINT('Ctrl Pts',(19.4316533015979,-20.9509276719108,-5.84825266693107));
#86640=CARTESIAN_POINT('Ctrl Pts',(19.4573309949732,-20.9417799062435,-5.84655092824721));
#86641=CARTESIAN_POINT('Ctrl Pts',(19.5312424694622,-20.9138290236909,-5.84155577834798));
#86642=CARTESIAN_POINT('Ctrl Pts',(19.578970470398,-20.8937499469217,-5.83820916551103));
#86643=CARTESIAN_POINT('Ctrl Pts',(19.7513075146447,-20.813690644089,-5.8257878301129));
#86644=CARTESIAN_POINT('Ctrl Pts',(19.8707060636378,-20.7432872504515,-5.81654188506069));
#86645=CARTESIAN_POINT('Ctrl Pts',(20.0148044229229,-20.63807245764,-5.80498894382203));
#86646=CARTESIAN_POINT('Ctrl Pts',(20.0465448755708,-20.6134832342372,-5.80241428550193));
#86647=CARTESIAN_POINT('Ctrl Pts',(20.1232083782398,-20.5505233744019,-5.79612733501363));
#86648=CARTESIAN_POINT('Ctrl Pts',(20.1672630672117,-20.5111455858879,-5.79245394757114));
#86649=CARTESIAN_POINT('Ctrl Pts',(20.2183862453488,-20.4614489214751,-5.78811263181848));
#86650=CARTESIAN_POINT('Ctrl Pts',(20.227081720279,-20.4528482795876,-5.78737127448224));
#86651=CARTESIAN_POINT('Ctrl Pts',(20.2412892904811,-20.438549973334,-5.78615491197485));
#86652=CARTESIAN_POINT('Ctrl Pts',(20.2468446954101,-20.4328959310682,-5.78567799303401));
#86653=CARTESIAN_POINT('Ctrl Pts',(20.2568085952445,-20.42264053584,-5.7848201996241));
#86654=CARTESIAN_POINT('Ctrl Pts',(20.2612282972139,-20.4180502491288,-5.78443883663041));
#86655=CARTESIAN_POINT('Ctrl Pts',(20.2706324608343,-20.4081944405868,-5.78362547086898));
#86656=CARTESIAN_POINT('Ctrl Pts',(20.2756107432682,-20.4029231153759,-5.78319373834905));
#86657=CARTESIAN_POINT('Ctrl Pts',(20.28903055778,-20.3885663108431,-5.7820266843052));
#86658=CARTESIAN_POINT('Ctrl Pts',(20.2974195777854,-20.3794319720167,-5.78129361294003));
#86659=CARTESIAN_POINT('Ctrl Pts',(20.3401523099804,-20.3320739967788,-5.77754027536949));
#86660=CARTESIAN_POINT('Ctrl Pts',(20.3731779965723,-20.2926810217713,-5.7745755781199));
#86661=CARTESIAN_POINT('Ctrl Pts',(20.5101613572313,-20.1166487804733,-5.76191625201652));
#86662=CARTESIAN_POINT('Ctrl Pts',(20.5987105623636,-19.968863126292,-5.75281706380873));
#86663=CARTESIAN_POINT('Ctrl Pts',(20.7054048832317,-19.7288713900421,-5.7383926325167));
#86664=CARTESIAN_POINT('Ctrl Pts',(20.7369623533648,-19.6434506633284,-5.73330447001261));
#86665=CARTESIAN_POINT('Ctrl Pts',(20.7656829766929,-19.5470181719367,-5.72734303716419));
#86666=CARTESIAN_POINT('Ctrl Pts',(20.7683772552651,-19.5377401454468,-5.72676728004617));
#86667=CARTESIAN_POINT('Ctrl Pts',(20.7722639615859,-19.5240055092786,-5.72591128899053));
#86668=CARTESIAN_POINT('Ctrl Pts',(20.7735055232919,-19.5195627712275,-5.72563383591011));
#86669=CARTESIAN_POINT('Ctrl Pts',(20.7756834930981,-19.5116698088704,-5.72513985160232));
#86670=CARTESIAN_POINT('Ctrl Pts',(20.7766256925935,-19.5082212335887,-5.72492366015826));
#86671=CARTESIAN_POINT('Ctrl Pts',(20.7786269157219,-19.5008228290067,-5.72445906327036));
#86672=CARTESIAN_POINT('Ctrl Pts',(20.7796832157756,-19.4968723723711,-5.72421051002225));
#86673=CARTESIAN_POINT('Ctrl Pts',(20.7825541577406,-19.4860093072181,-5.72352577079516));
#86674=CARTESIAN_POINT('Ctrl Pts',(20.7843452312957,-19.4790906056236,-5.72308825843168));
#86675=CARTESIAN_POINT('Ctrl Pts',(20.7937630546606,-19.4419362450744,-5.72073174931013));
#86676=CARTESIAN_POINT('Ctrl Pts',(20.8007556579683,-19.4115456201891,-5.71877941676331));
#86677=CARTESIAN_POINT('Ctrl Pts',(20.840282190576,-19.2205460098615,-5.70640137008781));
#86678=CARTESIAN_POINT('Ctrl Pts',(20.8547462255173,-19.0567703334592,-5.69536346719755));
#86679=CARTESIAN_POINT('Ctrl Pts',(20.8469095587802,-18.7758460519865,-5.67700415240263));
#86680=CARTESIAN_POINT('Ctrl Pts',(20.8339246690935,-18.6591838884141,-5.66953964958673));
#86681=CARTESIAN_POINT('Ctrl Pts',(20.8085934934435,-18.5301526884317,-5.6615105742519));
#86682=CARTESIAN_POINT('Ctrl Pts',(20.805697852025,-18.5161544505642,-5.66064231408016));
#86683=CARTESIAN_POINT('Ctrl Pts',(20.8008639251029,-18.4939235691392,-5.65926764211037));
#86684=CARTESIAN_POINT('Ctrl Pts',(20.799017742708,-18.4856715460704,-5.65875829983431));
#86685=CARTESIAN_POINT('Ctrl Pts',(20.7956746903455,-18.4711381037897,-5.65786282672941));
#86686=CARTESIAN_POINT('Ctrl Pts',(20.7941984407228,-18.4648520981111,-5.65747603933531));
#86687=CARTESIAN_POINT('Ctrl Pts',(20.7910857799759,-18.4518653486167,-5.65667798879759));
#86688=CARTESIAN_POINT('Ctrl Pts',(20.7894453320078,-18.4451656438717,-5.65626686080514));
#86689=CARTESIAN_POINT('Ctrl Pts',(20.7851508737915,-18.4279905856371,-5.65521432865093));
#86690=CARTESIAN_POINT('Ctrl Pts',(20.7824493271382,-18.4175272372723,-5.65457446476992));
#86691=CARTESIAN_POINT('Ctrl Pts',(20.770843162559,-18.3739564942231,-5.65191520729823));
#86692=CARTESIAN_POINT('Ctrl Pts',(20.7612148074383,-18.341046086698,-5.64991931067721));
#86693=CARTESIAN_POINT('Ctrl Pts',(20.7340522132623,-18.2559314289023,-5.6447791213387));
#86694=CARTESIAN_POINT('Ctrl Pts',(20.7152729622998,-18.2041508144812,-5.64167413957681));
#86695=CARTESIAN_POINT('Ctrl Pts',(20.6532485698303,-18.0519322729142,-5.63253422564439));
#86696=CARTESIAN_POINT('Ctrl Pts',(20.6042229019265,-17.9540500155665,-5.62664803774175));
#86697=CARTESIAN_POINT('Ctrl Pts',(20.5264211001456,-17.8247715683042,-5.61843346120246));
#86698=CARTESIAN_POINT('Ctrl Pts',(20.5039401887055,-17.7897913711027,-5.61616121667305));
#86699=CARTESIAN_POINT('Ctrl Pts',(20.436937111708,-17.6919920922932,-5.60960384701895));
#86700=CARTESIAN_POINT('Ctrl Pts',(20.3900029976483,-17.6309148007828,-5.60525832414802));
#86701=CARTESIAN_POINT('Ctrl Pts',(20.3336587858995,-17.5653236990881,-5.6001337453355));
#86702=CARTESIAN_POINT('Ctrl Pts',(20.3274151160633,-17.5581536472439,-5.59956703565788));
#86703=CARTESIAN_POINT('Ctrl Pts',(20.3180906160939,-17.5475901867729,-5.59872197520079));
#86704=CARTESIAN_POINT('Ctrl Pts',(20.3150466220836,-17.5441642207356,-5.59844630372645));
#86705=CARTESIAN_POINT('Ctrl Pts',(20.3096103236611,-17.5380856222539,-5.59795427608276));
#86706=CARTESIAN_POINT('Ctrl Pts',(20.3072224064655,-17.5354291337211,-5.59773824960221));
#86707=CARTESIAN_POINT('Ctrl Pts',(20.3020732722935,-17.5297299502232,-5.59727262132433));
#86708=CARTESIAN_POINT('Ctrl Pts',(20.2993099578999,-17.5266892911335,-5.59702286444327));
#86709=CARTESIAN_POINT('Ctrl Pts',(20.2916561865217,-17.5183164387628,-5.5963314867647));
#86710=CARTESIAN_POINT('Ctrl Pts',(20.286747272054,-17.5130013013145,-5.59588849744779));
#86711=CARTESIAN_POINT('Ctrl Pts',(20.2596762709581,-17.4839899218357,-5.59344849065966));
#86712=CARTESIAN_POINT('Ctrl Pts',(20.2370002093771,-17.4607817809088,-5.59141533965383));
#86713=CARTESIAN_POINT('Ctrl Pts',(20.0973946205978,-17.3243201436816,-5.57901130615425));
#86714=CARTESIAN_POINT('Ctrl Pts',(19.9682564581952,-17.224343344445,-5.56804903287148));
#86715=CARTESIAN_POINT('Ctrl Pts',(19.7289491046462,-17.0797247201609,-5.54978483409524));
#86716=CARTESIAN_POINT('Ctrl Pts',(19.6241159203917,-17.0276715710751,-5.5423426912471));
#86717=CARTESIAN_POINT('Ctrl Pts',(19.5022235771501,-16.979254248858,-5.53433426529295));
#86718=CARTESIAN_POINT('Ctrl Pts',(19.4888876693982,-16.9741127723112,-5.53346612179614));
#86719=CARTESIAN_POINT('Ctrl Pts',(19.4675807762464,-16.9661450866604,-5.53209159905664));
#86720=CARTESIAN_POINT('Ctrl Pts',(19.4596433378722,-16.9632309733015,-5.53158229032558));
#86721=CARTESIAN_POINT('Ctrl Pts',(19.445614076855,-16.9581755101072,-5.53068685624182));
#86722=CARTESIAN_POINT('Ctrl Pts',(19.4395295571149,-16.9560143446546,-5.53030007450372));
#86723=CARTESIAN_POINT('Ctrl Pts',(19.4269248010237,-16.9516020898591,-5.52950201653108));
#86724=CARTESIAN_POINT('Ctrl Pts',(19.4204032523089,-16.9493549601288,-5.52909087554189));
#86725=CARTESIAN_POINT('Ctrl Pts',(19.403636055677,-16.9436690142584,-5.52803827057667));
#86726=CARTESIAN_POINT('Ctrl Pts',(19.3933747674154,-16.9402766795595,-5.52739834729997));
#86727=CARTESIAN_POINT('Ctrl Pts',(19.3504470503807,-16.9264487161243,-5.52473851277569));
#86728=CARTESIAN_POINT('Ctrl Pts',(19.3175543898468,-16.9167286569075,-5.52274211151668));
#86729=CARTESIAN_POINT('Ctrl Pts',(19.2312560780637,-16.8934911086931,-5.51760032892731));
#86730=CARTESIAN_POINT('Ctrl Pts',(19.1775324962696,-16.8812508524518,-5.51449429051936));
#86731=CARTESIAN_POINT('Ctrl Pts',(19.0159317184782,-16.8510109383415,-5.50535253296559));
#86732=CARTESIAN_POINT('Ctrl Pts',(18.9070747335003,-16.8392561551318,-5.49946555200795));
#86733=CARTESIAN_POINT('Ctrl Pts',(18.7544605181739,-16.8346549291794,-5.49115293314775));
#86734=CARTESIAN_POINT('Ctrl Pts',(18.7110949416286,-16.8346800090703,-5.48878282590522));
#86735=CARTESIAN_POINT('Ctrl Pts',(18.6387105333112,-16.8369459271424,-5.48477287328617));
#86736=CARTESIAN_POINT('Ctrl Pts',(18.609681810146,-16.8384535272548,-5.48315018718292));
#86737=CARTESIAN_POINT('Ctrl Pts',(18.5332498328724,-16.8440030323251,-5.47881882376279));
#86738=CARTESIAN_POINT('Ctrl Pts',(18.4859387752249,-16.8490457142325,-5.47607786768121));
#86739=CARTESIAN_POINT('Ctrl Pts',(18.4311994456352,-16.8567529054084,-5.47279571767541));
#86740=CARTESIAN_POINT('Ctrl Pts',(18.4235631836976,-16.8578706959467,-5.47233532576442));
#86741=CARTESIAN_POINT('Ctrl Pts',(18.4113502443046,-16.8597266849239,-5.47159471656187));
#86742=CARTESIAN_POINT('Ctrl Pts',(18.4067695021204,-16.8604382174673,-5.47131596666438));
#86743=CARTESIAN_POINT('Ctrl Pts',(18.3986487575679,-16.8617269534771,-5.47082002294523));
#86744=CARTESIAN_POINT('Ctrl Pts',(18.3951078424171,-16.8622981145192,-5.47060317371342));
#86745=CARTESIAN_POINT('Ctrl Pts',(18.3875923628475,-16.8635299901456,-5.47014162029549));
#86746=CARTESIAN_POINT('Ctrl Pts',(18.3836182901994,-16.8641930429397,-5.46989679120201));
#86747=CARTESIAN_POINT('Ctrl Pts',(18.3728684132865,-16.866018159407,-5.46923249741576));
#86748=CARTESIAN_POINT('Ctrl Pts',(18.3660964059549,-16.8672018791504,-5.46881183252056));
#86749=CARTESIAN_POINT('Ctrl Pts',(18.3321381477671,-16.8733082529736,-5.46669184182298));
#86750=CARTESIAN_POINT('Ctrl Pts',(18.305045705954,-16.8787295469509,-5.46496647039749));
#86751=CARTESIAN_POINT('Ctrl Pts',(18.2264894029349,-16.8960545205585,-5.45987935058538));
#86752=CARTESIAN_POINT('Ctrl Pts',(18.1753572570648,-16.9093555495304,-5.45646222863149));
#86753=CARTESIAN_POINT('Ctrl Pts',(17.9780377817643,-16.9686473861364,-5.44298624312623));
#86754=CARTESIAN_POINT('Ctrl Pts',(17.8364985171484,-17.0285486237564,-5.4327301261204));
#86755=CARTESIAN_POINT('Ctrl Pts',(17.6322178904866,-17.1425049328573,-5.41770539632465));
#86756=CARTESIAN_POINT('Ctrl Pts',(17.564067935396,-17.1858012940929,-5.41264115752182));
#86757=CARTESIAN_POINT('Ctrl Pts',(17.4877006222605,-17.2406831648322,-5.40690597723646));
#86758=CARTESIAN_POINT('Ctrl Pts',(17.4769266843766,-17.2485816305824,-5.40609527355976));
#86759=CARTESIAN_POINT('Ctrl Pts',(17.4596757886423,-17.261481221151,-5.40479444163929));
#86760=CARTESIAN_POINT('Ctrl Pts',(17.4531519315467,-17.2664187454273,-5.40430185271708));
#86761=CARTESIAN_POINT('Ctrl Pts',(17.4417172321457,-17.2751777185676,-5.40343726363277));
#86762=CARTESIAN_POINT('Ctrl Pts',(17.4367943395821,-17.2789832064612,-5.40306464167132));
#86763=CARTESIAN_POINT('Ctrl Pts',(17.4265674645179,-17.286961050281,-5.40228968678376));
#86764=CARTESIAN_POINT('Ctrl Pts',(17.4212665039761,-17.2911371793684,-5.40188750945744));
#86765=CARTESIAN_POINT('Ctrl Pts',(17.4076756771347,-17.3019498332582,-5.40085506336682));
#86766=CARTESIAN_POINT('Ctrl Pts',(17.3994155483161,-17.3086235642033,-5.40022629044215));
#86767=CARTESIAN_POINT('Ctrl Pts',(17.3815453160414,-17.3232853298586,-5.39886295215658));
#86768=CARTESIAN_POINT('Ctrl Pts',(17.3719549823574,-17.3312969029837,-5.39812935681644));
#86769=CARTESIAN_POINT('Ctrl Pts',(17.3443462413243,-17.3547788528114,-5.39601124820017));
#86770=CARTESIAN_POINT('Ctrl Pts',(17.326516177287,-17.3704683643157,-5.39463555590603));
#86771=CARTESIAN_POINT('Ctrl Pts',(17.2657069690694,-17.4258203083558,-5.38991087557279));
#86772=CARTESIAN_POINT('Ctrl Pts',(17.2241082658136,-17.4669624325992,-5.38662114313595));
#86773=CARTESIAN_POINT('Ctrl Pts',(17.0705437080051,-17.6319746888536,-5.37412048580666));
#86774=CARTESIAN_POINT('Ctrl Pts',(16.9716851432441,-17.7671822761984,-5.36533072763668));
#86775=CARTESIAN_POINT('Ctrl Pts',(16.861928867705,-17.9619260508484,-5.35279259969752));
#86776=CARTESIAN_POINT('Ctrl Pts',(16.8361147496659,-18.0123579789408,-5.34955027416261));
#86777=CARTESIAN_POINT('Ctrl Pts',(16.8086439393009,-18.0717890596408,-5.34566589901993));
#86778=CARTESIAN_POINT('Ctrl Pts',(16.8049826228568,-18.0798422089399,-5.34513823146));
#86779=CARTESIAN_POINT('Ctrl Pts',(16.7995310102159,-18.0920354248045,-5.34433696023719));
#86780=CARTESIAN_POINT('Ctrl Pts',(16.7977032434327,-18.096158769006,-5.34406559602872));
#86781=CARTESIAN_POINT('Ctrl Pts',(16.7944540629059,-18.1035524333439,-5.34357823553818));
#86782=CARTESIAN_POINT('Ctrl Pts',(16.7930277230357,-18.1068205307497,-5.34336254449328));
#86783=CARTESIAN_POINT('Ctrl Pts',(16.7899554460828,-18.1139086722036,-5.34289413450356));
#86784=CARTESIAN_POINT('Ctrl Pts',(16.7883125308254,-18.1177299160629,-5.34264124174425));
#86785=CARTESIAN_POINT('Ctrl Pts',(16.7837517930946,-18.1284244493725,-5.34193248465295));
#86786=CARTESIAN_POINT('Ctrl Pts',(16.7808590919814,-18.135308292111,-5.34147513874715));
#86787=CARTESIAN_POINT('Ctrl Pts',(16.7642159201089,-18.1755086922632,-5.33879834044752));
#86788=CARTESIAN_POINT('Ctrl Pts',(16.7512825491522,-18.2091546432478,-5.33653418196317));
#86789=CARTESIAN_POINT('Ctrl Pts',(16.7123640076299,-18.3186699693303,-5.32912522136634));
#86790=CARTESIAN_POINT('Ctrl Pts',(16.6898292561938,-18.3956877983485,-5.32385730482946));
#86791=CARTESIAN_POINT('Ctrl Pts',(16.6354452693788,-18.6302199152264,-5.30796210733017));
#86792=CARTESIAN_POINT('Ctrl Pts',(16.6170836152047,-18.7902875361735,-5.29735395519403));
#86793=CARTESIAN_POINT('Ctrl Pts',(16.617000284924,-18.950901652078,-5.287306223149));
#86794=CARTESIAN_POINT('Ctrl Pts',(16.6170002837517,-18.9509039138869,-5.28730608165431));
#86795=CARTESIAN_POINT('Ctrl Pts',(16.6169868618986,-18.9768271136034,-5.28568437341906));
#86796=CARTESIAN_POINT('Ctrl Pts',(16.6174495936726,-19.0027494402333,-5.28407668181815));
#86797=CARTESIAN_POINT('Ctrl Pts',(16.6190263323593,-19.0462644316672,-5.28140090717751));
#86798=CARTESIAN_POINT('Ctrl Pts',(16.6198840725923,-19.0638627409736,-5.2803250904963));
#86799=CARTESIAN_POINT('Ctrl Pts',(16.6214584306178,-19.0895615601323,-5.27876299448743));
#86800=CARTESIAN_POINT('Ctrl Pts',(16.622002162565,-19.0976715578003,-5.27827132879577));
#86801=CARTESIAN_POINT('Ctrl Pts',(16.6230473372594,-19.1120220182355,-5.27740358485186));
#86802=CARTESIAN_POINT('Ctrl Pts',(16.6235297763737,-19.1182637277103,-5.27702691438678));
#86803=CARTESIAN_POINT('Ctrl Pts',(16.6245388687493,-19.1306063621236,-5.27628352984855));
#86804=CARTESIAN_POINT('Ctrl Pts',(16.6250643197426,-19.1367073214785,-5.27591678175321));
#86805=CARTESIAN_POINT('Ctrl Pts',(16.6261638694004,-19.1488572175267,-5.27518778927124));
#86806=CARTESIAN_POINT('Ctrl Pts',(16.6267375530475,-19.1549061319947,-5.27482553551552));
#86807=CARTESIAN_POINT('Ctrl Pts',(16.628171445051,-19.1693626531271,-5.27396135880791));
#86808=CARTESIAN_POINT('Ctrl Pts',(16.6290559778645,-19.1777677847624,-5.27346020459241));
#86809=CARTESIAN_POINT('Ctrl Pts',(16.6319011557525,-19.2033318817324,-5.27193970815204));
#86810=CARTESIAN_POINT('Ctrl Pts',(16.6340214891345,-19.2204726163725,-5.27092537975229));
#86811=CARTESIAN_POINT('Ctrl Pts',(16.6419662055849,-19.2788271263581,-5.2674880714534));
#86812=CARTESIAN_POINT('Ctrl Pts',(16.6487962825489,-19.3198955704463,-5.26509633678038));
#86813=CARTESIAN_POINT('Ctrl Pts',(16.6780901110545,-19.4687639697274,-5.2564924142788));
#86814=CARTESIAN_POINT('Ctrl Pts',(16.7077221576998,-19.5748697951031,-5.25049678246115));
#86815=CARTESIAN_POINT('Ctrl Pts',(16.7454193808392,-19.6781102678644,-5.2445270093495));
#86816=CARTESIAN_POINT('Origin',(18.734,-18.952,0.));
#86817=CARTESIAN_POINT('',(16.7454194481082,-19.6781104520924,-4.44630497675564));
#86818=CARTESIAN_POINT('',(16.7454194642264,-19.6781104962347,-4.66702132639115));
#86819=CARTESIAN_POINT('',(16.7454194499637,-19.6781104571739,0.));
#86820=CARTESIAN_POINT('Ctrl Pts',(16.7454194642264,-19.6781104962347,-4.66702132639115));
#86821=CARTESIAN_POINT('Ctrl Pts',(16.6988234569433,-19.5504991841709,-4.67446196791304));
#86822=CARTESIAN_POINT('Ctrl Pts',(16.6646102515307,-19.4186749085756,-4.68169548970326));
#86823=CARTESIAN_POINT('Ctrl Pts',(16.6370543933824,-19.2453826839987,-4.69152883179162));
#86824=CARTESIAN_POINT('Ctrl Pts',(16.6319381922759,-19.2061457568985,-4.69377780195413));
#86825=CARTESIAN_POINT('Ctrl Pts',(16.626393980434,-19.1517834673221,-4.69695245069132));
#86826=CARTESIAN_POINT('Ctrl Pts',(16.6250239200878,-19.1367604804233,-4.69783593480563));
#86827=CARTESIAN_POINT('Ctrl Pts',(16.6229323255952,-19.1107556897743,-4.69937787446987));
#86828=CARTESIAN_POINT('Ctrl Pts',(16.6221356455221,-19.0997803490558,-4.70003253407433));
#86829=CARTESIAN_POINT('Ctrl Pts',(16.6211102620138,-19.083945503156,-4.70098328869644));
#86830=CARTESIAN_POINT('Ctrl Pts',(16.6208126722558,-19.0790904303007,-4.70127564097596));
#86831=CARTESIAN_POINT('Ctrl Pts',(16.6203235174173,-19.0706328035693,-4.70178646094323));
#86832=CARTESIAN_POINT('Ctrl Pts',(16.6201244222697,-19.0670306778377,-4.70200450695554));
#86833=CARTESIAN_POINT('Ctrl Pts',(16.6197264096993,-19.0594793959756,-4.70246265010531));
#86834=CARTESIAN_POINT('Ctrl Pts',(16.6195293494743,-19.0555302017514,-4.70270284534969));
#86835=CARTESIAN_POINT('Ctrl Pts',(16.6190357978485,-19.045049313883,-4.70334184113573));
#86836=CARTESIAN_POINT('Ctrl Pts',(16.6187585035133,-19.0385168200452,-4.7037416930887));
#86837=CARTESIAN_POINT('Ctrl Pts',(16.6177066685289,-19.0106966833973,-4.70545098301501));
#86838=CARTESIAN_POINT('Ctrl Pts',(16.6172232246242,-18.9894001117826,-4.7067754745818));
#86839=CARTESIAN_POINT('Ctrl Pts',(16.6170218767854,-18.9629268972801,-4.70843883518829));
#86840=CARTESIAN_POINT('Ctrl Pts',(16.617001493557,-18.9577528772316,-4.70876473205849));
#86841=CARTESIAN_POINT('Ctrl Pts',(16.6169868171325,-18.9040721310964,-4.71215391963486));
#86842=CARTESIAN_POINT('Ctrl Pts',(16.6186407108799,-18.8555823846155,-4.71528276307785));
#86843=CARTESIAN_POINT('Ctrl Pts',(16.6353861336127,-18.6113422023217,-4.73125347287945));
#86844=CARTESIAN_POINT('Ctrl Pts',(16.6759975092691,-18.4182600520973,-4.74444611234127));
#86845=CARTESIAN_POINT('Ctrl Pts',(16.7587957195953,-18.188768490955,-4.75978160671345));
#86846=CARTESIAN_POINT('Ctrl Pts',(16.7764544949314,-18.1445531266853,-4.7627263938696));
#86847=CARTESIAN_POINT('Ctrl Pts',(16.8006203664839,-18.08951013166,-4.76638234636621));
#86848=CARTESIAN_POINT('Ctrl Pts',(16.8057522333939,-18.078097178512,-4.76713987196758));
#86849=CARTESIAN_POINT('Ctrl Pts',(16.8140577650559,-18.0600556036716,-4.76833670074756));
#86850=CARTESIAN_POINT('Ctrl Pts',(16.8171652099536,-18.0533969833946,-4.76877827062177));
#86851=CARTESIAN_POINT('Ctrl Pts',(16.8230280562325,-18.0410029007359,-4.76959996751399));
#86852=CARTESIAN_POINT('Ctrl Pts',(16.8257747611383,-18.0352634381284,-4.76998038978466));
#86853=CARTESIAN_POINT('Ctrl Pts',(16.8319433130545,-18.0225215979931,-4.7708247836726));
#86854=CARTESIAN_POINT('Ctrl Pts',(16.8353780473832,-18.0155255349562,-4.77128830088787));
#86855=CARTESIAN_POINT('Ctrl Pts',(16.8455036892124,-17.9951857541092,-4.77263568882129));
#86856=CARTESIAN_POINT('Ctrl Pts',(16.8522972741185,-17.9818934669447,-4.77351596196072));
#86857=CARTESIAN_POINT('Ctrl Pts',(16.9092402191692,-17.873328397997,-4.78070598899491));
#86858=CARTESIAN_POINT('Ctrl Pts',(16.9664529930495,-17.7819304747911,-4.78674994189988));
#86859=CARTESIAN_POINT('Ctrl Pts',(17.109755897751,-17.5876688993976,-4.80001598495269));
#86860=CARTESIAN_POINT('Ctrl Pts',(17.199144359828,-17.4878335212404,-4.80713503285765));
#86861=CARTESIAN_POINT('Ctrl Pts',(17.3093993042227,-17.385963236324,-4.81548117151138));
#86862=CARTESIAN_POINT('Ctrl Pts',(17.3215810198652,-17.3749676945156,-4.81639828677522));
#86863=CARTESIAN_POINT('Ctrl Pts',(17.3736914804033,-17.3290195133269,-4.82030637030103));
#86864=CARTESIAN_POINT('Ctrl Pts',(17.4147958908763,-17.2954359528519,-4.82335194662809));
#86865=CARTESIAN_POINT('Ctrl Pts',(17.4640568970095,-17.2581849938948,-4.82701707861956));
#86866=CARTESIAN_POINT('Ctrl Pts',(17.4710315783227,-17.2529780696824,-4.82753635589282));
#86867=CARTESIAN_POINT('Ctrl Pts',(17.4816442233066,-17.2451566924231,-4.82832733821555));
#86868=CARTESIAN_POINT('Ctrl Pts',(17.4852588009897,-17.2425104606685,-4.82859688852883));
#86869=CARTESIAN_POINT('Ctrl Pts',(17.4917638953347,-17.2377797222716,-4.82908231315701));
#86870=CARTESIAN_POINT('Ctrl Pts',(17.4946512981478,-17.2356910257103,-4.82929789256426));
#86871=CARTESIAN_POINT('Ctrl Pts',(17.5009390259754,-17.2311667343445,-4.82976760828476));
#86872=CARTESIAN_POINT('Ctrl Pts',(17.5043412547042,-17.2287339545885,-4.8300219268285));
#86873=CARTESIAN_POINT('Ctrl Pts',(17.5139238827321,-17.2219246780926,-4.83073862991125));
#86874=CARTESIAN_POINT('Ctrl Pts',(17.5201205163407,-17.2175712910091,-4.83120254904962));
#86875=CARTESIAN_POINT('Ctrl Pts',(17.5574250787705,-17.1916611531595,-4.83399750136794));
#86876=CARTESIAN_POINT('Ctrl Pts',(17.5890811189297,-17.170909955644,-4.83637787189424));
#86877=CARTESIAN_POINT('Ctrl Pts',(17.6953691754556,-17.1052404387069,-4.84435477389429));
#86878=CARTESIAN_POINT('Ctrl Pts',(17.7722144513456,-17.0640801112438,-4.85009442603247));
#86879=CARTESIAN_POINT('Ctrl Pts',(18.0107217372933,-16.9546785314189,-4.86743165257851));
#86880=CARTESIAN_POINT('Ctrl Pts',(18.1785690169876,-16.9016477585081,-4.87894119187821));
#86881=CARTESIAN_POINT('Ctrl Pts',(18.3736798159472,-16.8657623757734,-4.89115217917399));
#86882=CARTESIAN_POINT('Ctrl Pts',(18.3963686451636,-16.8619705280759,-4.89255633845765));
#86883=CARTESIAN_POINT('Ctrl Pts',(18.4285570947284,-16.8571289318122,-4.89452678066019));
#86884=CARTESIAN_POINT('Ctrl Pts',(18.4380083163656,-16.8557726534075,-4.89510272231644));
#86885=CARTESIAN_POINT('Ctrl Pts',(18.4533807096104,-16.8536727089882,-4.89603531575576));
#86886=CARTESIAN_POINT('Ctrl Pts',(18.4592963408922,-16.8528900678741,-4.8963931957589));
#86887=CARTESIAN_POINT('Ctrl Pts',(18.4716866918103,-16.8513040929079,-4.89714071219739));
#86888=CARTESIAN_POINT('Ctrl Pts',(18.4781619836584,-16.8505056563029,-4.89753019028512));
#86889=CARTESIAN_POINT('Ctrl Pts',(18.4935765002678,-16.848677269474,-4.89845459190866));
#86890=CARTESIAN_POINT('Ctrl Pts',(18.5025188505678,-16.847674348102,-4.89898865816394));
#86891=CARTESIAN_POINT('Ctrl Pts',(18.5326724272337,-16.8444870381601,-4.90078231527588));
#86892=CARTESIAN_POINT('Ctrl Pts',(18.5539106200222,-16.8425660617114,-4.9020336227825));
#86893=CARTESIAN_POINT('Ctrl Pts',(18.6697220741529,-16.8338529005574,-4.90879683995305));
#86894=CARTESIAN_POINT('Ctrl Pts',(18.7646461587201,-16.833098720746,-4.91411557334995));
#86895=CARTESIAN_POINT('Ctrl Pts',(19.0284689899736,-16.8487424624775,-4.92865727462931));
#86896=CARTESIAN_POINT('Ctrl Pts',(19.1957911698045,-16.8790451841467,-4.93757429016926));
#86897=CARTESIAN_POINT('Ctrl Pts',(19.3942326978688,-16.9402237222502,-4.94941731566111));
#86898=CARTESIAN_POINT('Ctrl Pts',(19.4304574451852,-16.9524756501796,-4.95163587933073));
#86899=CARTESIAN_POINT('Ctrl Pts',(19.4731106509165,-16.9682014457571,-4.95433801193991));
#86900=CARTESIAN_POINT('Ctrl Pts',(19.4798803577023,-16.9707368305246,-4.95476961075706));
#86901=CARTESIAN_POINT('Ctrl Pts',(19.4908791616161,-16.9749204528084,-4.95547548944941));
#86902=CARTESIAN_POINT('Ctrl Pts',(19.4951162413002,-16.9765477308828,-4.95574854562345));
#86903=CARTESIAN_POINT('Ctrl Pts',(19.5026747936992,-16.9794785696899,-4.956237728215));
#86904=CARTESIAN_POINT('Ctrl Pts',(19.5059982336508,-16.9807769130603,-4.95645353977999));
#86905=CARTESIAN_POINT('Ctrl Pts',(19.513169763893,-16.9835994793816,-4.95692080598098));
#86906=CARTESIAN_POINT('Ctrl Pts',(19.5170166171156,-16.9851265655413,-4.95717242687282));
#86907=CARTESIAN_POINT('Ctrl Pts',(19.5277035002433,-16.9894052605318,-4.95787411954539));
#86908=CARTESIAN_POINT('Ctrl Pts',(19.5345335938311,-16.9921813045193,-4.95832562646303));
#86909=CARTESIAN_POINT('Ctrl Pts',(19.5732653755652,-17.0081598172767,-4.96090279374959));
#86910=CARTESIAN_POINT('Ctrl Pts',(19.6048528720404,-17.0221046702017,-4.96306943810205));
#86911=CARTESIAN_POINT('Ctrl Pts',(19.7036616063405,-17.0686451715156,-4.97002246954352));
#86912=CARTESIAN_POINT('Ctrl Pts',(19.7695035696544,-17.1040281752955,-4.97491682217222));
#86913=CARTESIAN_POINT('Ctrl Pts',(19.9992014125371,-17.2436016448319,-4.99264425422368));
#86914=CARTESIAN_POINT('Ctrl Pts',(20.1504628739279,-17.3667479439259,-5.00547037846406));
#86915=CARTESIAN_POINT('Ctrl Pts',(20.2972373612967,-17.5242659670621,-5.01869782342656));
#86916=CARTESIAN_POINT('Ctrl Pts',(20.3114107851474,-17.5399409423562,-5.01998620073653));
#86917=CARTESIAN_POINT('Ctrl Pts',(20.330821585278,-17.5620652108692,-5.02176686976182));
#86918=CARTESIAN_POINT('Ctrl Pts',(20.33625893219,-17.5683366700919,-5.02226749857302));
#86919=CARTESIAN_POINT('Ctrl Pts',(20.3455867507635,-17.5792241320495,-5.02312956967299));
#86920=CARTESIAN_POINT('Ctrl Pts',(20.3494945922022,-17.5838250614038,-5.02349172823265));
#86921=CARTESIAN_POINT('Ctrl Pts',(20.3575518636169,-17.5933940072849,-5.02424054430023));
#86922=CARTESIAN_POINT('Ctrl Pts',(20.3616982994939,-17.5983644713011,-5.02462707676828));
#86923=CARTESIAN_POINT('Ctrl Pts',(20.3713655994835,-17.6100616186339,-5.02553108681136));
#86924=CARTESIAN_POINT('Ctrl Pts',(20.3768679401055,-17.6168035123711,-5.02604780861657));
#86925=CARTESIAN_POINT('Ctrl Pts',(20.3946413288914,-17.6388570557911,-5.02772424372196));
#86926=CARTESIAN_POINT('Ctrl Pts',(20.4067413295677,-17.6543056994098,-5.02887710028773));
#86927=CARTESIAN_POINT('Ctrl Pts',(20.4677836211424,-17.7345139826193,-5.03475724037706));
#86928=CARTESIAN_POINT('Ctrl Pts',(20.5131895213832,-17.8018849723305,-5.0393452707916));
#86929=CARTESIAN_POINT('Ctrl Pts',(20.6406534510727,-18.0166992390387,-5.0531884414534));
#86930=CARTESIAN_POINT('Ctrl Pts',(20.7090523841095,-18.1714391576291,-5.0620596615006));
#86931=CARTESIAN_POINT('Ctrl Pts',(20.7741179477669,-18.3841053186586,-5.07456202087068));
#86932=CARTESIAN_POINT('Ctrl Pts',(20.7878941317968,-18.4361478299142,-5.07764924545969));
#86933=CARTESIAN_POINT('Ctrl Pts',(20.8015839524154,-18.4971792190701,-5.08136089540101));
#86934=CARTESIAN_POINT('Ctrl Pts',(20.803443475616,-18.5057164149007,-5.08188214256367));
#86935=CARTESIAN_POINT('Ctrl Pts',(20.8061778320212,-18.5186546814733,-5.08267554156417));
#86936=CARTESIAN_POINT('Ctrl Pts',(20.8070916340495,-18.5230475450693,-5.08294551891231));
#86937=CARTESIAN_POINT('Ctrl Pts',(20.8087062463014,-18.5309350462942,-5.08343139760595));
#86938=CARTESIAN_POINT('Ctrl Pts',(20.8094122021839,-18.5344285756738,-5.08364700160978));
#86939=CARTESIAN_POINT('Ctrl Pts',(20.8109263507429,-18.5420202673165,-5.08411640228897));
#86940=CARTESIAN_POINT('Ctrl Pts',(20.8117312271716,-18.5461189896515,-5.08437037918332));
#86941=CARTESIAN_POINT('Ctrl Pts',(20.813956401713,-18.5576304608555,-5.08508517552231));
#86942=CARTESIAN_POINT('Ctrl Pts',(20.8153491785127,-18.5650483756389,-5.08554751676513));
#86943=CARTESIAN_POINT('Ctrl Pts',(20.823407876091,-18.6092715464762,-5.08831349690364));
#86944=CARTESIAN_POINT('Ctrl Pts',(20.8291366281751,-18.6462383650756,-5.09066531570909));
#86945=CARTESIAN_POINT('Ctrl Pts',(20.8447157358734,-18.7680043940224,-5.09850005886564));
#86946=CARTESIAN_POINT('Ctrl Pts',(20.8504170577727,-18.8532464401609,-5.10412098239));
#86947=CARTESIAN_POINT('Ctrl Pts',(20.8520835937592,-19.1164030776585,-5.12150613993781));
#86948=CARTESIAN_POINT('Ctrl Pts',(20.8308029983747,-19.293684130979,-5.13319015950719));
#86949=CARTESIAN_POINT('Ctrl Pts',(20.7820535464246,-19.4883635979075,-5.14554080955071));
#86950=CARTESIAN_POINT('Ctrl Pts',(20.77615573115,-19.5103988465163,-5.14693304107251));
#86951=CARTESIAN_POINT('Ctrl Pts',(20.7672940952352,-19.5414867933826,-5.14888980255299));
#86952=CARTESIAN_POINT('Ctrl Pts',(20.7646237123329,-19.5506208322699,-5.14946381034992));
#86953=CARTESIAN_POINT('Ctrl Pts',(20.7601804364233,-19.5654471265633,-5.15039412793865));
#86954=CARTESIAN_POINT('Ctrl Pts',(20.7584449504504,-19.5711503708782,-5.15075165409909));
#86955=CARTESIAN_POINT('Ctrl Pts',(20.7547582186108,-19.5830846644017,-5.15149911026087));
#86956=CARTESIAN_POINT('Ctrl Pts',(20.7528021871447,-19.5893141787053,-5.15188887893397));
#86957=CARTESIAN_POINT('Ctrl Pts',(20.7480735952767,-19.6041334380661,-5.15281520608287));
#86958=CARTESIAN_POINT('Ctrl Pts',(20.7452748449081,-19.6127147420156,-5.15335089764109));
#86959=CARTESIAN_POINT('Ctrl Pts',(20.735628094291,-19.6416634590871,-5.15515583012444));
#86960=CARTESIAN_POINT('Ctrl Pts',(20.728524774723,-19.6619448483473,-5.15641664286948));
#86961=CARTESIAN_POINT('Ctrl Pts',(20.6593009910564,-19.8503473638225,-5.16810322495215));
#86962=CARTESIAN_POINT('Ctrl Pts',(20.5763775377804,-20.0100472139787,-5.1777344611722));
#86963=CARTESIAN_POINT('Ctrl Pts',(20.4055670582364,-20.2566572969864,-5.19406000301463));
#86964=CARTESIAN_POINT('Ctrl Pts',(20.328463064136,-20.3498362250276,-5.20068308558403));
#86965=CARTESIAN_POINT('Ctrl Pts',(20.2372032464848,-20.4426907926725,-5.20839927507256));
#86966=CARTESIAN_POINT('Ctrl Pts',(20.2305066482437,-20.4494133977567,-5.20896488448912));
#86967=CARTESIAN_POINT('Ctrl Pts',(20.2205117239458,-20.4593131275309,-5.20980861478114));
#86968=CARTESIAN_POINT('Ctrl Pts',(20.2172478112813,-20.4625250409313,-5.21008406857941));
#86969=CARTESIAN_POINT('Ctrl Pts',(20.2114196428091,-20.4682232540697,-5.21057585819148));
#86970=CARTESIAN_POINT('Ctrl Pts',(20.2088594909027,-20.4707136790727,-5.21079186555056));
#86971=CARTESIAN_POINT('Ctrl Pts',(20.2033388703169,-20.4760568184924,-5.21125762451018));
#86972=CARTESIAN_POINT('Ctrl Pts',(20.2003764340119,-20.4789073498178,-5.21150753210191));
#86973=CARTESIAN_POINT('Ctrl Pts',(20.1921695041917,-20.486758354533,-5.21219974206957));
#86974=CARTESIAN_POINT('Ctrl Pts',(20.1869076680303,-20.4917405023072,-5.21264341828775));
#86975=CARTESIAN_POINT('Ctrl Pts',(20.157828151169,-20.518992542863,-5.21509414724068));
#86976=CARTESIAN_POINT('Ctrl Pts',(20.1335253562638,-20.5407355789536,-5.21713770126414));
#86977=CARTESIAN_POINT('Ctrl Pts',(19.9850465325458,-20.6675245929747,-5.22954523903706));
#86978=CARTESIAN_POINT('Ctrl Pts',(19.8496058956549,-20.758534107256,-5.24049798826835));
#86979=CARTESIAN_POINT('Ctrl Pts',(19.6012651554108,-20.886732643794,-5.25875317507815));
#86980=CARTESIAN_POINT('Ctrl Pts',(19.4931765863139,-20.9316459216739,-5.26619530806575));
#86981=CARTESIAN_POINT('Ctrl Pts',(19.3683368794992,-20.9717794926344,-5.27420197547602));
#86982=CARTESIAN_POINT('Ctrl Pts',(19.3547128580724,-20.9760079147617,-5.27506842114454));
#86983=CARTESIAN_POINT('Ctrl Pts',(19.3329543038577,-20.9825206472383,-5.27644077215336));
#86984=CARTESIAN_POINT('Ctrl Pts',(19.3248472203679,-20.9848944690724,-5.27694959259776));
#86985=CARTESIAN_POINT('Ctrl Pts',(19.3105198928001,-20.9889966831563,-5.27784445889519));
#86986=CARTESIAN_POINT('Ctrl Pts',(19.3043055850123,-20.9907452550821,-5.27823115851425));
#86987=CARTESIAN_POINT('Ctrl Pts',(19.2914318144341,-20.9943041879194,-5.27902932567515));
#86988=CARTESIAN_POINT('Ctrl Pts',(19.284771295619,-20.9961104680013,-5.27944065659752));
#86989=CARTESIAN_POINT('Ctrl Pts',(19.2676435156226,-21.0006655936315,-5.28049432519043));
#86990=CARTESIAN_POINT('Ctrl Pts',(19.2571637116441,-21.0033668257279,-5.28113511604412));
#86991=CARTESIAN_POINT('Ctrl Pts',(19.2132663224012,-21.0143233618144,-5.28380339296977));
#86992=CARTESIAN_POINT('Ctrl Pts',(19.1796695204334,-21.0218436495487,-5.28580717813392));
#86993=CARTESIAN_POINT('Ctrl Pts',(19.091597778484,-21.0393135599577,-5.29097229240118));
#86994=CARTESIAN_POINT('Ctrl Pts',(19.0368886497974,-21.0479516186433,-5.294093808669));
#86995=CARTESIAN_POINT('Ctrl Pts',(18.8730940357218,-21.0672648340811,-5.3032625605962));
#86996=CARTESIAN_POINT('Ctrl Pts',(18.7634527245879,-21.0716287091711,-5.30916115023632));
#86997=CARTESIAN_POINT('Ctrl Pts',(18.593661112367,-21.0652051429016,-5.31841310948858));
#86998=CARTESIAN_POINT('Ctrl Pts',(18.5334831769926,-21.0603461124867,-5.32171765286354));
#86999=CARTESIAN_POINT('Ctrl Pts',(18.4157969663717,-21.0457593265224,-5.32836057403453));
#87000=CARTESIAN_POINT('Ctrl Pts',(18.3583215465393,-21.0362134478195,-5.33169108892318));
#87001=CARTESIAN_POINT('Ctrl Pts',(18.2926015762768,-21.0224916636395,-5.33567374155975));
#87002=CARTESIAN_POINT('Ctrl Pts',(18.2838963721323,-21.0206166913074,-5.33620485123954));
#87003=CARTESIAN_POINT('Ctrl Pts',(18.2707881091677,-21.0177067071606,-5.33701034022951));
#87004=CARTESIAN_POINT('Ctrl Pts',(18.2663759881435,-21.0167123863822,-5.33728244488949));
#87005=CARTESIAN_POINT('Ctrl Pts',(18.2584901017543,-21.0149086404725,-5.33777060092777));
#87006=CARTESIAN_POINT('Ctrl Pts',(18.2550151659508,-21.0141045683352,-5.33798634285901));
#87007=CARTESIAN_POINT('Ctrl Pts',(18.2475010769315,-21.0123458504461,-5.33845424385345));
#87008=CARTESIAN_POINT('Ctrl Pts',(18.2434627499495,-21.01138812059,-5.33870657338992));
#87009=CARTESIAN_POINT('Ctrl Pts',(18.2322075486001,-21.0086838526422,-5.339412199354));
#87010=CARTESIAN_POINT('Ctrl Pts',(18.2249970902658,-21.0069112312037,-5.33986695669133));
#87011=CARTESIAN_POINT('Ctrl Pts',(18.1835029577228,-20.9964785100172,-5.34249899316209));
#87012=CARTESIAN_POINT('Ctrl Pts',(18.1494333585219,-20.9869989860733,-5.34471928541359));
#87013=CARTESIAN_POINT('Ctrl Pts',(18.0413221830518,-20.9539793880848,-5.3519209300234));
#87014=CARTESIAN_POINT('Ctrl Pts',(17.9683350467338,-20.9272163355083,-5.35701840454586));
#87015=CARTESIAN_POINT('Ctrl Pts',(17.7269462436826,-20.8233107164373,-5.37436203939018));
#87016=CARTESIAN_POINT('Ctrl Pts',(17.5672000795249,-20.728109757915,-5.38658232570517));
#87017=CARTESIAN_POINT('Ctrl Pts',(17.4024685262322,-20.5980023674751,-5.39952483469995));
#87018=CARTESIAN_POINT('Ctrl Pts',(17.383342064452,-20.5823444672028,-5.4010353085623));
#87019=CARTESIAN_POINT('Ctrl Pts',(17.3569924000674,-20.5599912406533,-5.40312803996645));
#87020=CARTESIAN_POINT('Ctrl Pts',(17.3495356163368,-20.5535755167236,-5.40372163285419));
#87021=CARTESIAN_POINT('Ctrl Pts',(17.3375875035354,-20.5431497053441,-5.40467505580946));
#87022=CARTESIAN_POINT('Ctrl Pts',(17.3330681556735,-20.5391720807194,-5.40503622395731));
#87023=CARTESIAN_POINT('Ctrl Pts',(17.3240140414579,-20.5311344600123,-5.40576090779376));
#87024=CARTESIAN_POINT('Ctrl Pts',(17.3194796934778,-20.5270740775325,-5.40612440227856));
#87025=CARTESIAN_POINT('Ctrl Pts',(17.3087651588247,-20.5173959242197,-5.40698472385317));
#87026=CARTESIAN_POINT('Ctrl Pts',(17.302600550861,-20.5117609983964,-5.40748082081452));
#87027=CARTESIAN_POINT('Ctrl Pts',(17.2834008785157,-20.4940013303064,-5.409029561869));
#87028=CARTESIAN_POINT('Ctrl Pts',(17.2704850889812,-20.4817483609572,-5.41007672649453));
#87029=CARTESIAN_POINT('Ctrl Pts',(17.240760746323,-20.4528283529638,-5.41250045665302));
#87030=CARTESIAN_POINT('Ctrl Pts',(17.2240739439454,-20.4360392792182,-5.41387168165147));
#87031=CARTESIAN_POINT('Ctrl Pts',(17.1673425623045,-20.377012502134,-5.41857620144597));
#87032=CARTESIAN_POINT('Ctrl Pts',(17.12875902556,-20.3334044712007,-5.42185082491593));
#87033=CARTESIAN_POINT('Ctrl Pts',(16.9876329321103,-20.1599902756054,-5.43425259867397));
#87034=CARTESIAN_POINT('Ctrl Pts',(16.8986446806635,-20.0199432858701,-5.44296640652934));
#87035=CARTESIAN_POINT('Ctrl Pts',(16.8014676033383,-19.8182737938716,-5.45550400786095));
#87036=CARTESIAN_POINT('Ctrl Pts',(16.7782692661977,-19.7645439925457,-5.45884882988038));
#87037=CARTESIAN_POINT('Ctrl Pts',(16.7541361330696,-19.7016049160798,-5.46284742918434));
#87038=CARTESIAN_POINT('Ctrl Pts',(16.7509973612087,-19.6932617554037,-5.46337908118137));
#87039=CARTESIAN_POINT('Ctrl Pts',(16.7470769047147,-19.6826376833051,-5.46405840735278));
#87040=CARTESIAN_POINT('Ctrl Pts',(16.7462462413202,-19.6803747699851,-5.46420323660037));
#87041=CARTESIAN_POINT('Ctrl Pts',(16.7454194499637,-19.6781104571738,-5.46434829365948));
#87042=CARTESIAN_POINT('Ctrl Pts',(16.7454193808392,-19.6781102678644,-5.2445270093495));
#87043=CARTESIAN_POINT('Ctrl Pts',(16.766587520815,-19.7360829405597,-5.24117479976143));
#87044=CARTESIAN_POINT('Ctrl Pts',(16.7902987735039,-19.7931519605987,-5.23782816634432));
#87045=CARTESIAN_POINT('Ctrl Pts',(16.8430672133903,-19.905935431496,-5.23098482781489));
#87046=CARTESIAN_POINT('Ctrl Pts',(16.8721437371547,-19.9615096429608,-5.22749298686203));
#87047=CARTESIAN_POINT('Ctrl Pts',(16.9191780065077,-20.0424431844216,-5.22210863640132));
#87048=CARTESIAN_POINT('Ctrl Pts',(16.9352983718101,-20.0688336636703,-5.2203028337863));
#87049=CARTESIAN_POINT('Ctrl Pts',(16.9558380198731,-20.1008602101464,-5.21803690875092));
#87050=CARTESIAN_POINT('Ctrl Pts',(16.9597163425328,-20.1068408156888,-5.21761051028791));
#87051=CARTESIAN_POINT('Ctrl Pts',(16.9658647109005,-20.1162178867387,-5.21693661732211));
#87052=CARTESIAN_POINT('Ctrl Pts',(16.9681145521302,-20.1196276258782,-5.21669045477579));
#87053=CARTESIAN_POINT('Ctrl Pts',(16.972352171989,-20.1260096745917,-5.21622756624743));
#87054=CARTESIAN_POINT('Ctrl Pts',(16.9743376167184,-20.1289834672395,-5.21601099645364));
#87055=CARTESIAN_POINT('Ctrl Pts',(16.9789053705132,-20.135787642143,-5.21551346204761));
#87056=CARTESIAN_POINT('Ctrl Pts',(16.9814926820624,-20.1396146006955,-5.21523216255377));
#87057=CARTESIAN_POINT('Ctrl Pts',(16.9895487918989,-20.1514469463241,-5.21435795785947));
#87058=CARTESIAN_POINT('Ctrl Pts',(16.9950599823428,-20.1594231243758,-5.21376228682459));
#87059=CARTESIAN_POINT('Ctrl Pts',(17.057328512786,-20.2482318608905,-5.20706090588122));
#87060=CARTESIAN_POINT('Ctrl Pts',(17.1196150892808,-20.3250262359966,-5.20062764184388));
#87061=CARTESIAN_POINT('Ctrl Pts',(17.3015407196668,-20.5197658748576,-5.18307319119865));
#87062=CARTESIAN_POINT('Ctrl Pts',(17.4302426709673,-20.6283241836233,-5.17192748815693));
#87063=CARTESIAN_POINT('Ctrl Pts',(17.5967906935513,-20.7379003696934,-5.15940133548108));
#87064=CARTESIAN_POINT('Ctrl Pts',(17.6235431142517,-20.7546565971322,-5.15743871609121));
#87065=CARTESIAN_POINT('Ctrl Pts',(17.663828306338,-20.7786516966939,-5.15455519329351));
#87066=CARTESIAN_POINT('Ctrl Pts',(17.6770802753552,-20.7863512722429,-5.15361788548105));
#87067=CARTESIAN_POINT('Ctrl Pts',(17.7013526902698,-20.8001035066598,-5.15192118619002));
#87068=CARTESIAN_POINT('Ctrl Pts',(17.7123455763817,-20.8062031407082,-5.1511601327394));
#87069=CARTESIAN_POINT('Ctrl Pts',(17.7297375582689,-20.815651816551,-5.14996744860832));
#87070=CARTESIAN_POINT('Ctrl Pts',(17.7361004400565,-20.8190665803556,-5.14953347771465));
#87071=CARTESIAN_POINT('Ctrl Pts',(17.7425268617856,-20.8224732072189,-5.14909753375409));
#87072=CARTESIAN_POINT('Ctrl Pts',(17.7425729938427,-20.8224976594978,-5.14909440445328));
#87073=CARTESIAN_POINT('Ctrl Pts',(17.7426668840093,-20.8225474214947,-5.14908803579943));
#87074=CARTESIAN_POINT('Ctrl Pts',(17.7427146432438,-20.8225727316523,-5.14908479637879));
#87075=CARTESIAN_POINT('Ctrl Pts',(17.7428118470268,-20.8226242403368,-5.14907820349224));
#87076=CARTESIAN_POINT('Ctrl Pts',(17.7428612926443,-20.8226504392621,-5.14907484996318));
#87077=CARTESIAN_POINT('Ctrl Pts',(17.7429619308434,-20.8227037576371,-5.14906802470699));
#87078=CARTESIAN_POINT('Ctrl Pts',(17.743013124214,-20.8227308773245,-5.1490645529364));
#87079=CARTESIAN_POINT('Ctrl Pts',(17.743117321722,-20.8227860704755,-5.14905748690083));
#87080=CARTESIAN_POINT('Ctrl Pts',(17.7431703266561,-20.8228141441677,-5.14905389259261));
#87081=CARTESIAN_POINT('Ctrl Pts',(17.7432782133937,-20.8228712797516,-5.14904657703208));
#87082=CARTESIAN_POINT('Ctrl Pts',(17.7433330959254,-20.8229003418214,-5.14904285574198));
#87083=CARTESIAN_POINT('Ctrl Pts',(17.7434448063247,-20.822959489785,-5.14903528161055));
#87084=CARTESIAN_POINT('Ctrl Pts',(17.743501634972,-20.8229895758691,-5.14903142872876));
#87085=CARTESIAN_POINT('Ctrl Pts',(17.7436173086067,-20.8230508087759,-5.14902358663774));
#87086=CARTESIAN_POINT('Ctrl Pts',(17.743676154301,-20.8230819557338,-5.14901959739391));
#87087=CARTESIAN_POINT('Ctrl Pts',(17.7437959355681,-20.823145348586,-5.14901147763401));
#87088=CARTESIAN_POINT('Ctrl Pts',(17.743856871888,-20.8231775946193,-5.1490073470816));
#87089=CARTESIAN_POINT('Ctrl Pts',(17.7439809106413,-20.8232432251852,-5.14899893958042));
#87090=CARTESIAN_POINT('Ctrl Pts',(17.7440440137244,-20.8232766097863,-5.14899466260297));
#87091=CARTESIAN_POINT('Ctrl Pts',(17.7441724650629,-20.8233445584779,-5.14898595693991));
#87092=CARTESIAN_POINT('Ctrl Pts',(17.7442378137746,-20.8233791225145,-5.14898152823984));
#87093=CARTESIAN_POINT('Ctrl Pts',(17.7443708402382,-20.8234494735391,-5.14897251349784));
#87094=CARTESIAN_POINT('Ctrl Pts',(17.7444385152684,-20.8234852587705,-5.1489679276581));
#87095=CARTESIAN_POINT('Ctrl Pts',(17.7445651243489,-20.8235521983873,-5.14895934878097));
#87096=CARTESIAN_POINT('Ctrl Pts',(17.7446240593062,-20.8235833543873,-5.14895535561881));
#87097=CARTESIAN_POINT('Ctrl Pts',(17.7447516802526,-20.8236508135633,-5.14894670903985));
#87098=CARTESIAN_POINT('Ctrl Pts',(17.7448203678529,-20.8236871163154,-5.14894205558503));
#87099=CARTESIAN_POINT('Ctrl Pts',(17.7449690906242,-20.8237657087608,-5.14893198048351));
#87100=CARTESIAN_POINT('Ctrl Pts',(17.7450491272721,-20.8238079975053,-5.14892655883323));
#87101=CARTESIAN_POINT('Ctrl Pts',(17.7452223979139,-20.823899533824,-5.14891482234299));
#87102=CARTESIAN_POINT('Ctrl Pts',(17.7453156337355,-20.8239487800211,-5.14890850750991));
#87103=CARTESIAN_POINT('Ctrl Pts',(17.7455174428088,-20.8240553542039,-5.14889484012024));
#87104=CARTESIAN_POINT('Ctrl Pts',(17.7456260178439,-20.8241126799613,-5.14888748761968));
#87105=CARTESIAN_POINT('Ctrl Pts',(17.7458609760584,-20.8242367077338,-5.14887157814187));
#87106=CARTESIAN_POINT('Ctrl Pts',(17.7459873606819,-20.824303406227,-5.14886302130579));
#87107=CARTESIAN_POINT('Ctrl Pts',(17.7462732878129,-20.8244542650139,-5.1488436647522));
#87108=CARTESIAN_POINT('Ctrl Pts',(17.7464328343613,-20.8245384177338,-5.14883286530239));
#87109=CARTESIAN_POINT('Ctrl Pts',(17.7523042955182,-20.8276343568583,-5.14843548898989));
#87110=CARTESIAN_POINT('Ctrl Pts',(17.7580299975305,-20.8306200394255,-5.14804983972057));
#87111=CARTESIAN_POINT('Ctrl Pts',(17.7712868466837,-20.8374558928897,-5.14716118240317));
#87112=CARTESIAN_POINT('Ctrl Pts',(17.7788276184615,-20.8412872371119,-5.14665884156104));
#87113=CARTESIAN_POINT('Ctrl Pts',(17.7991802191402,-20.8514750637132,-5.14531132592591));
#87114=CARTESIAN_POINT('Ctrl Pts',(17.8120339736784,-20.8577471504928,-5.14446909880766));
#87115=CARTESIAN_POINT('Ctrl Pts',(17.9304952245364,-20.9140721555885,-5.13678484369134));
#87116=CARTESIAN_POINT('Ctrl Pts',(18.0400204122868,-20.9554332195214,-5.1302596633236));
#87117=CARTESIAN_POINT('Ctrl Pts',(18.3090878571133,-21.0323099481725,-5.11494052932477));
#87118=CARTESIAN_POINT('Ctrl Pts',(18.4703872106178,-21.0588308344687,-5.1063302845368));
#87119=CARTESIAN_POINT('Ctrl Pts',(18.6653454802484,-21.0681325740938,-5.09512043216081));
#87120=CARTESIAN_POINT('Ctrl Pts',(18.6976103034938,-21.0689331704703,-5.09323780193555));
#87121=CARTESIAN_POINT('Ctrl Pts',(18.7371021885638,-21.069010050594,-5.09088632858741));
#87122=CARTESIAN_POINT('Ctrl Pts',(18.7443255076406,-21.0689871417563,-5.09045429818655));
#87123=CARTESIAN_POINT('Ctrl Pts',(18.755654446319,-21.0688932295526,-5.08977348372276));
#87124=CARTESIAN_POINT('Ctrl Pts',(18.7597602956431,-21.0688472469408,-5.08952607756281));
#87125=CARTESIAN_POINT('Ctrl Pts',(18.7674380497953,-21.0687389209107,-5.08906215353391));
#87126=CARTESIAN_POINT('Ctrl Pts',(18.7710099394135,-21.0686794812152,-5.08884579970967));
#87127=CARTESIAN_POINT('Ctrl Pts',(18.7791677093746,-21.0685230727996,-5.0883504847758));
#87128=CARTESIAN_POINT('Ctrl Pts',(18.7837534202208,-21.0684202408607,-5.08807119994708));
#87129=CARTESIAN_POINT('Ctrl Pts',(18.7978633104379,-21.0680579518034,-5.08720930749281));
#87130=CARTESIAN_POINT('Ctrl Pts',(18.8073859477431,-21.0677491043806,-5.08662404296766));
#87131=CARTESIAN_POINT('Ctrl Pts',(18.9364094484131,-21.0626924060164,-5.0786486255935));
#87132=CARTESIAN_POINT('Ctrl Pts',(19.0552876961205,-21.0478911239382,-5.07078168182625));
#87133=CARTESIAN_POINT('Ctrl Pts',(19.2788786405678,-21.0005779722052,-5.05568356514402));
#87134=CARTESIAN_POINT('Ctrl Pts',(19.3835995988073,-20.969817702043,-5.04848028866793));
#87135=CARTESIAN_POINT('Ctrl Pts',(19.555649795197,-20.9044887718609,-5.0366556435896));
#87136=CARTESIAN_POINT('Ctrl Pts',(19.6243473337719,-20.8741354173499,-5.03193410381107));
#87137=CARTESIAN_POINT('Ctrl Pts',(19.7080706811158,-20.8316885625777,-5.02618365802385));
#87138=CARTESIAN_POINT('Ctrl Pts',(19.724733240119,-20.8229597715777,-5.02503922898156));
#87139=CARTESIAN_POINT('Ctrl Pts',(19.7488019061056,-20.8099395234349,-5.02338571777478));
#87140=CARTESIAN_POINT('Ctrl Pts',(19.7563014684108,-20.8058235871889,-5.02287043898416));
#87141=CARTESIAN_POINT('Ctrl Pts',(19.7694107919308,-20.798525137866,-5.02196955171942));
#87142=CARTESIAN_POINT('Ctrl Pts',(19.7750313038117,-20.7953622592235,-5.02158324725687));
#87143=CARTESIAN_POINT('Ctrl Pts',(19.7859200928922,-20.7891690324963,-5.0208347014047));
#87144=CARTESIAN_POINT('Ctrl Pts',(19.7911899411518,-20.7861415881294,-5.02047236046221));
#87145=CARTESIAN_POINT('Ctrl Pts',(19.8037616307306,-20.7788471680432,-5.01960776213131));
#87146=CARTESIAN_POINT('Ctrl Pts',(19.8110511200237,-20.7745590278453,-5.01910627520533));
#87147=CARTESIAN_POINT('Ctrl Pts',(19.8372914704912,-20.7589103788829,-5.01730026903631));
#87148=CARTESIAN_POINT('Ctrl Pts',(19.8560903088074,-20.7472967941979,-5.01600497276923));
#87149=CARTESIAN_POINT('Ctrl Pts',(20.0311434415229,-20.6353281251975,-5.0039191883543));
#87150=CARTESIAN_POINT('Ctrl Pts',(20.1737332115338,-20.51512154638,-4.99398657516972));
#87151=CARTESIAN_POINT('Ctrl Pts',(20.3527449112073,-20.3186617741078,-4.97949715573226));
#87152=CARTESIAN_POINT('Ctrl Pts',(20.4032658492327,-20.2564726959617,-4.97509385549669));
#87153=CARTESIAN_POINT('Ctrl Pts',(20.4712245579586,-20.1623869300008,-4.96845482327554));
#87154=CARTESIAN_POINT('Ctrl Pts',(20.4915597685408,-20.1326646420797,-4.96636025103566));
#87155=CARTESIAN_POINT('Ctrl Pts',(20.5151824756617,-20.0961738130957,-4.96377331908926));
#87156=CARTESIAN_POINT('Ctrl Pts',(20.5192059329232,-20.0898859782372,-4.96332701873268));
#87157=CARTESIAN_POINT('Ctrl Pts',(20.5254190746871,-20.0800620535029,-4.96262868054329));
#87158=CARTESIAN_POINT('Ctrl Pts',(20.5276317819882,-20.0765404962315,-4.96237814003187));
#87159=CARTESIAN_POINT('Ctrl Pts',(20.5317223407796,-20.0699875228954,-4.96191149810616));
#87160=CARTESIAN_POINT('Ctrl Pts',(20.5336029155269,-20.0669578744101,-4.96169558017775));
#87161=CARTESIAN_POINT('Ctrl Pts',(20.5378451202764,-20.0600848931543,-4.96120536547796));
#87162=CARTESIAN_POINT('Ctrl Pts',(20.5402021141446,-20.0562387741653,-4.96093077104908));
#87163=CARTESIAN_POINT('Ctrl Pts',(20.5462565768015,-20.0462879142601,-4.96021969089374));
#87164=CARTESIAN_POINT('Ctrl Pts',(20.5499354633916,-20.0401720125702,-4.95978203778065));
#87165=CARTESIAN_POINT('Ctrl Pts',(20.5723483959082,-20.0024818317104,-4.95708172441507));
#87166=CARTESIAN_POINT('Ctrl Pts',(20.5902881748598,-19.9704452565031,-4.9547727560753));
#87167=CARTESIAN_POINT('Ctrl Pts',(20.6867179231991,-19.7872229537487,-4.94155886630472));
#87168=CARTESIAN_POINT('Ctrl Pts',(20.7475683369636,-19.627463017674,-4.93006552004989));
#87169=CARTESIAN_POINT('Ctrl Pts',(20.8116276936537,-19.3694572989089,-4.91278865567016));
#87170=CARTESIAN_POINT('Ctrl Pts',(20.8283436721875,-19.2753207036624,-4.90672137455992));
#87171=CARTESIAN_POINT('Ctrl Pts',(20.8409557520772,-19.1590859664567,-4.899539592127));
#87172=CARTESIAN_POINT('Ctrl Pts',(20.8429418766939,-19.1377723129207,-4.89823491464743));
#87173=CARTESIAN_POINT('Ctrl Pts',(20.8453044509209,-19.1074468728523,-4.89639535026117));
#87174=CARTESIAN_POINT('Ctrl Pts',(20.8459470550914,-19.098457690731,-4.89585214384242));
#87175=CARTESIAN_POINT('Ctrl Pts',(20.846956051088,-19.0829516109355,-4.89491864504823));
#87176=CARTESIAN_POINT('Ctrl Pts',(20.8473497378375,-19.0764366718422,-4.8945275010291));
#87177=CARTESIAN_POINT('Ctrl Pts',(20.8480455105541,-19.0639649575464,-4.89378073307569));
#87178=CARTESIAN_POINT('Ctrl Pts',(20.848352563931,-19.0580085323544,-4.89342495695304));
#87179=CARTESIAN_POINT('Ctrl Pts',(20.8490849375401,-19.0425293776329,-4.89250262481711));
#87180=CARTESIAN_POINT('Ctrl Pts',(20.8494711243088,-19.0330048637839,-4.89193729946376));
#87181=CARTESIAN_POINT('Ctrl Pts',(20.8505663600304,-19.0005851852725,-4.89002026297689));
#87182=CARTESIAN_POINT('Ctrl Pts',(20.8509681706519,-18.9776807583392,-4.88867816039968));
#87183=CARTESIAN_POINT('Ctrl Pts',(20.851229575852,-18.7781617034181,-4.87708341780581));
#87184=CARTESIAN_POINT('Ctrl Pts',(20.829361441651,-18.602217347693,-4.8675930135609));
#87185=CARTESIAN_POINT('Ctrl Pts',(20.7646769364804,-18.3474564016516,-4.85328877317991));
#87186=CARTESIAN_POINT('Ctrl Pts',(20.7383771435592,-18.2652746547204,-4.84856656756729));
#87187=CARTESIAN_POINT('Ctrl Pts',(20.6935117335157,-18.1498664672737,-4.84149553779059));
#87188=CARTESIAN_POINT('Ctrl Pts',(20.6789483711616,-18.1151727309016,-4.83930983139501));
#87189=CARTESIAN_POINT('Ctrl Pts',(20.6603586326572,-18.0739973946479,-4.83662183706322));
#87190=CARTESIAN_POINT('Ctrl Pts',(20.6572108943854,-18.0671237327015,-4.83616991467182));
#87191=CARTESIAN_POINT('Ctrl Pts',(20.6522658375635,-18.0564763281121,-4.83546467867024));
#87192=CARTESIAN_POINT('Ctrl Pts',(20.6504940094967,-18.0526907198608,-4.83521291061632));
#87193=CARTESIAN_POINT('Ctrl Pts',(20.6471906361685,-18.0456869791504,-4.83474516617037));
#87194=CARTESIAN_POINT('Ctrl Pts',(20.645662170996,-18.0424674577108,-4.83452938075615));
#87195=CARTESIAN_POINT('Ctrl Pts',(20.6421925719484,-18.0352065614768,-4.83404099001893));
#87196=CARTESIAN_POINT('Ctrl Pts',(20.6402467364802,-18.0311675074361,-4.83376809652335));
#87197=CARTESIAN_POINT('Ctrl Pts',(20.6344781796465,-18.0192901083543,-4.83296210202507));
#87198=CARTESIAN_POINT('Ctrl Pts',(20.6306198911076,-18.0114692796454,-4.83242686389385));
#87199=CARTESIAN_POINT('Ctrl Pts',(20.602809084369,-17.9559632462738,-4.82859708094487));
#87200=CARTESIAN_POINT('Ctrl Pts',(20.5771114118441,-17.9091788767439,-4.82520540835786));
#87201=CARTESIAN_POINT('Ctrl Pts',(20.5406308361121,-17.8483318014866,-4.82062024229572));
#87202=CARTESIAN_POINT('Ctrl Pts',(20.5313974494874,-17.8333575840296,-4.81947726885003));
#87203=CARTESIAN_POINT('Ctrl Pts',(20.4960067582514,-17.7775324149195,-4.81516533873204));
#87204=CARTESIAN_POINT('Ctrl Pts',(20.4686350687213,-17.7374701054467,-4.81196761509608));
#87205=CARTESIAN_POINT('Ctrl Pts',(20.3751395338638,-17.6102419595451,-4.80153801718461));
#87206=CARTESIAN_POINT('Ctrl Pts',(20.3036277226784,-17.5272453240315,-4.79430521460465));
#87207=CARTESIAN_POINT('Ctrl Pts',(20.1869268550375,-17.4113090083487,-4.78373155890178));
#87208=CARTESIAN_POINT('Ctrl Pts',(20.1463327209863,-17.3740132180049,-4.78024232864403));
#87209=CARTESIAN_POINT('Ctrl Pts',(20.0781788869175,-17.3161366592632,-4.77468462779284));
#87210=CARTESIAN_POINT('Ctrl Pts',(20.0514942741945,-17.2945698194499,-4.77257771618738));
#87211=CARTESIAN_POINT('Ctrl Pts',(20.0157271243577,-17.267072285667,-4.7698411375673));
#87212=CARTESIAN_POINT('Ctrl Pts',(20.0071077824445,-17.2605502062117,-4.76918812816274));
#87213=CARTESIAN_POINT('Ctrl Pts',(19.9929062908602,-17.2499742852708,-4.76812262252011));
#87214=CARTESIAN_POINT('Ctrl Pts',(19.9873536860634,-17.2458812696209,-4.76770859680545));
#87215=CARTESIAN_POINT('Ctrl Pts',(19.9765651572319,-17.2380097668315,-4.76690908102986));
#87216=CARTESIAN_POINT('Ctrl Pts',(19.9713317639453,-17.2342279555421,-4.76652346461807));
#87217=CARTESIAN_POINT('Ctrl Pts',(19.9592058925206,-17.2255495949808,-4.76563504748775));
#87218=CARTESIAN_POINT('Ctrl Pts',(19.9523011902965,-17.2206702529721,-4.76513291281909));
#87219=CARTESIAN_POINT('Ctrl Pts',(19.9336483469028,-17.2076557000433,-4.76378631531194));
#87220=CARTESIAN_POINT('Ctrl Pts',(19.9218466341522,-17.1995977683016,-4.76294479379496));
#87221=CARTESIAN_POINT('Ctrl Pts',(19.8128225415864,-17.1267661589018,-4.75526373942634));
#87222=CARTESIAN_POINT('Ctrl Pts',(19.7104705291067,-17.0700203989717,-4.74874081322979));
#87223=CARTESIAN_POINT('Ctrl Pts',(19.4555786734846,-16.9551277701251,-4.73343476879697));
#87224=CARTESIAN_POINT('Ctrl Pts',(19.3000127977038,-16.9055904261853,-4.72483473639969));
#87225=CARTESIAN_POINT('Ctrl Pts',(19.1084259258384,-16.8681211455224,-4.71362572691807));
#87226=CARTESIAN_POINT('Ctrl Pts',(19.0763835274958,-16.8626175283382,-4.71172963484275));
#87227=CARTESIAN_POINT('Ctrl Pts',(19.0370676437198,-16.8567932282768,-4.70936318384116));
#87228=CARTESIAN_POINT('Ctrl Pts',(19.0299008439791,-16.8557690728276,-4.70893019320783));
#87229=CARTESIAN_POINT('Ctrl Pts',(19.0186577398976,-16.8542212078362,-4.70824819892432));
#87230=CARTESIAN_POINT('Ctrl Pts',(19.0145848458527,-16.8536725628841,-4.70800058107788));
#87231=CARTESIAN_POINT('Ctrl Pts',(19.006969077476,-16.8526692396113,-4.70753647822845));
#87232=CARTESIAN_POINT('Ctrl Pts',(19.0034266412007,-16.8522116670656,-4.7073201585988));
#87233=CARTESIAN_POINT('Ctrl Pts',(18.9953378568608,-16.8511876536293,-4.70682520975616));
#87234=CARTESIAN_POINT('Ctrl Pts',(18.9907908333071,-16.8506270066669,-4.70654625867494));
#87235=CARTESIAN_POINT('Ctrl Pts',(18.9768095792498,-16.8489491776177,-4.70568639621303));
#87236=CARTESIAN_POINT('Ctrl Pts',(18.9673697710596,-16.8478807553937,-4.70510284568251));
#87237=CARTESIAN_POINT('Ctrl Pts',(18.8825212210361,-16.8388553648033,-4.69983276152158));
#87238=CARTESIAN_POINT('Ctrl Pts',(18.8067505566895,-16.8348926292283,-4.69495155210683));
#87239=CARTESIAN_POINT('Ctrl Pts',(18.5460078963864,-16.8352695263499,-4.67789874624842));
#87240=CARTESIAN_POINT('Ctrl Pts',(18.361868355271,-16.8597698922016,-4.66550126466966));
#87241=CARTESIAN_POINT('Ctrl Pts',(18.1318242036018,-16.9217512133695,-4.65047365238472));
#87242=CARTESIAN_POINT('Ctrl Pts',(18.0809343291922,-16.9375442785673,-4.64717204959153));
#87243=CARTESIAN_POINT('Ctrl Pts',(18.0188622064967,-16.9594076673491,-4.64317035359587));
#87244=CARTESIAN_POINT('Ctrl Pts',(18.0070709027976,-16.9636790082869,-4.64241129965314));
#87245=CARTESIAN_POINT('Ctrl Pts',(17.9884946156015,-16.9705955144042,-4.64121706777149));
#87246=CARTESIAN_POINT('Ctrl Pts',(17.9816842705339,-16.9731712911504,-4.6407795860556));
#87247=CARTESIAN_POINT('Ctrl Pts',(17.968942136332,-16.9780658508525,-4.63996165395531));
#87248=CARTESIAN_POINT('Ctrl Pts',(17.9630072758027,-16.9803763593079,-4.63958093167464));
#87249=CARTESIAN_POINT('Ctrl Pts',(17.9497500584347,-16.9856065580718,-4.63873098233023));
#87250=CARTESIAN_POINT('Ctrl Pts',(17.9424333762112,-16.9885404455456,-4.63826223907311));
#87251=CARTESIAN_POINT('Ctrl Pts',(17.9239381222289,-16.9960769714797,-4.63707811788252));
#87252=CARTESIAN_POINT('Ctrl Pts',(17.9127821794531,-17.0007346567875,-4.63636460548998));
#87253=CARTESIAN_POINT('Ctrl Pts',(17.8493619227521,-17.0278533142955,-4.6323115959134));
#87254=CARTESIAN_POINT('Ctrl Pts',(17.7979771221796,-17.05231923767,-4.62904120507475));
#87255=CARTESIAN_POINT('Ctrl Pts',(17.7238770941782,-17.0913383529907,-4.62431038061396));
#87256=CARTESIAN_POINT('Ctrl Pts',(17.7003571218875,-17.104300749741,-4.62280633893005));
#87257=CARTESIAN_POINT('Ctrl Pts',(17.5767140127845,-17.1755433072049,-4.61486879543645));
#87258=CARTESIAN_POINT('Ctrl Pts',(17.4812554902167,-17.2415201802596,-4.60864385438076));
#87259=CARTESIAN_POINT('Ctrl Pts',(17.3297826760241,-17.3657249882551,-4.59796497741273));
#87260=CARTESIAN_POINT('Ctrl Pts',(17.2708254324822,-17.4199383530675,-4.59356323234316));
#87261=CARTESIAN_POINT('Ctrl Pts',(17.1900057647959,-17.5031843092151,-4.58692631508331));
#87262=CARTESIAN_POINT('Ctrl Pts',(17.1655927582505,-17.529648608672,-4.58483219916652));
#87263=CARTESIAN_POINT('Ctrl Pts',(17.1369482556436,-17.5623344126283,-4.5822457734869));
#87264=CARTESIAN_POINT('Ctrl Pts',(17.1320583318607,-17.567974130664,-4.58179950201406));
#87265=CARTESIAN_POINT('Ctrl Pts',(17.1244905661914,-17.5767961317317,-4.58110119927231));
#87266=CARTESIAN_POINT('Ctrl Pts',(17.1217920478787,-17.5799607092899,-4.58085066507877));
#87267=CARTESIAN_POINT('Ctrl Pts',(17.1167971340474,-17.5858533730527,-4.58038402877505));
#87268=CARTESIAN_POINT('Ctrl Pts',(17.1144982999495,-17.5885793169779,-4.58016811011205));
#87269=CARTESIAN_POINT('Ctrl Pts',(17.1093069064879,-17.5947668948988,-4.57967788578656));
#87270=CARTESIAN_POINT('Ctrl Pts',(17.1064185323918,-17.5982319566796,-4.57940328241668));
#87271=CARTESIAN_POINT('Ctrl Pts',(17.0978965089804,-17.608522166995,-4.57858763518222));
#87272=CARTESIAN_POINT('Ctrl Pts',(17.0922946398145,-17.6153733411435,-4.57804437860432));
#87273=CARTESIAN_POINT('Ctrl Pts',(17.0511025652341,-17.6664015011843,-4.5739979557316));
#87274=CARTESIAN_POINT('Ctrl Pts',(17.0172610927965,-17.7119542016744,-4.57038509107753));
#87275=CARTESIAN_POINT('Ctrl Pts',(16.9504035834435,-17.8099384376311,-4.56270239707196));
#87276=CARTESIAN_POINT('Ctrl Pts',(16.9177751688064,-17.8625746658577,-4.55862477889792));
#87277=CARTESIAN_POINT('Ctrl Pts',(16.8338945754426,-18.0121591752151,-4.54729667055912));
#87278=CARTESIAN_POINT('Ctrl Pts',(16.7877886608281,-18.1117820025346,-4.54004809148312));
#87279=CARTESIAN_POINT('Ctrl Pts',(16.730316654,-18.2664292459557,-4.52944127177649));
#87280=CARTESIAN_POINT('Ctrl Pts',(16.7130722623162,-18.3190654686249,-4.5259347676104));
#87281=CARTESIAN_POINT('Ctrl Pts',(16.6884846752926,-18.4054279846415,-4.52035278549321));
#87282=CARTESIAN_POINT('Ctrl Pts',(16.6798675390215,-18.4387613002577,-4.51823844646771));
#87283=CARTESIAN_POINT('Ctrl Pts',(16.6696144564368,-18.4828321771183,-4.51549378007866));
#87284=CARTESIAN_POINT('Ctrl Pts',(16.6672430078921,-18.4933916039965,-4.51483993742794));
#87285=CARTESIAN_POINT('Ctrl Pts',(16.6634921046792,-18.5107136083516,-4.513773420653));
#87286=CARTESIAN_POINT('Ctrl Pts',(16.662064583693,-18.5174654715133,-4.51335921144638));
#87287=CARTESIAN_POINT('Ctrl Pts',(16.6593656414592,-18.5305466191723,-4.51255958175244));
#87288=CARTESIAN_POINT('Ctrl Pts',(16.6580901071835,-18.5368749680149,-4.51217403365391));
#87289=CARTESIAN_POINT('Ctrl Pts',(16.6552123725028,-18.5514973710976,-4.51128611711599));
#87290=CARTESIAN_POINT('Ctrl Pts',(16.6536308208215,-18.5597954137541,-4.51078441231691));
#87291=CARTESIAN_POINT('Ctrl Pts',(16.6495122711773,-18.5821305926305,-4.50943972839927));
#87292=CARTESIAN_POINT('Ctrl Pts',(16.6470673798474,-18.5961844243212,-4.50859967738244));
#87293=CARTESIAN_POINT('Ctrl Pts',(16.6261906884283,-18.7238153608063,-4.50102301408465));
#87294=CARTESIAN_POINT('Ctrl Pts',(16.6169037095493,-18.8387007765424,-4.49459281209416));
#87295=CARTESIAN_POINT('Ctrl Pts',(16.6171578058381,-19.1400360565124,-4.47808638902454));
#87296=CARTESIAN_POINT('Ctrl Pts',(16.641892451733,-19.3254189864425,-4.46831880430488));
#87297=CARTESIAN_POINT('Ctrl Pts',(16.6942562459763,-19.5188655759305,-4.45654184705318));
#87298=CARTESIAN_POINT('Ctrl Pts',(16.6981093691169,-19.5325518735356,-4.45569945744374));
#87299=CARTESIAN_POINT('Ctrl Pts',(16.7036607300232,-19.5515351289403,-4.454516918222));
#87300=CARTESIAN_POINT('Ctrl Pts',(16.7052425224844,-19.556866115661,-4.45418327316907));
#87301=CARTESIAN_POINT('Ctrl Pts',(16.707815642707,-19.5654144473005,-4.45364567221952));
#87302=CARTESIAN_POINT('Ctrl Pts',(16.7087936865895,-19.568635809576,-4.45344248887362));
#87303=CARTESIAN_POINT('Ctrl Pts',(16.7108530770338,-19.575361030647,-4.45301703730184));
#87304=CARTESIAN_POINT('Ctrl Pts',(16.7119358439041,-19.5788644146348,-4.4527946835878));
#87305=CARTESIAN_POINT('Ctrl Pts',(16.7145777265088,-19.5873343839741,-4.45225538864194));
#87306=CARTESIAN_POINT('Ctrl Pts',(16.7161460644909,-19.5922980491595,-4.45193791126062));
#87307=CARTESIAN_POINT('Ctrl Pts',(16.7216994278518,-19.6096509575292,-4.45082311577179));
#87308=CARTESIAN_POINT('Ctrl Pts',(16.7257802847427,-19.6220089032853,-4.45002045156157));
#87309=CARTESIAN_POINT('Ctrl Pts',(16.7349633439441,-19.6489799213563,-4.44825062879185));
#87310=CARTESIAN_POINT('Ctrl Pts',(16.7401119394289,-19.6635749106904,-4.44728123477407));
#87311=CARTESIAN_POINT('Ctrl Pts',(16.7454194481082,-19.6781104520924,-4.44630497675564));
#87312=CARTESIAN_POINT('Origin',(18.734,-18.952,0.));
#87313=CARTESIAN_POINT('',(16.7454194499637,-19.6781104571739,-3.64442446316901));
#87314=CARTESIAN_POINT('',(16.7454195176904,-19.6781106426554,-3.86819360277559));
#87315=CARTESIAN_POINT('',(16.7454194499637,-19.6781104571739,0.));
#87316=CARTESIAN_POINT('',(16.6170009086013,-18.9500541448918,-3.91098515934228));
#87317=CARTESIAN_POINT('Ctrl Pts',(16.7454195176904,-19.6781106426554,-3.8681936027756));
#87318=CARTESIAN_POINT('Ctrl Pts',(16.734008174336,-19.6468586910403,-3.870273038502));
#87319=CARTESIAN_POINT('Ctrl Pts',(16.7233298307746,-19.615327548151,-3.87233004139765));
#87320=CARTESIAN_POINT('Ctrl Pts',(16.7086937631107,-19.5684998312811,-3.87532604665878));
#87321=CARTESIAN_POINT('Ctrl Pts',(16.7041601155389,-19.5534045723869,-3.87628296738397));
#87322=CARTESIAN_POINT('Ctrl Pts',(16.6975600376633,-19.5305036165196,-3.87772163856799));
#87323=CARTESIAN_POINT('Ctrl Pts',(16.6953690625293,-19.5227346652623,-3.87820743698151));
#87324=CARTESIAN_POINT('Ctrl Pts',(16.6915244726395,-19.5087975367014,-3.87907495627617));
#87325=CARTESIAN_POINT('Ctrl Pts',(16.6898542406799,-19.5026340824737,-3.87945721338924));
#87326=CARTESIAN_POINT('Ctrl Pts',(16.6863713150496,-19.48954719446,-3.88026595964412));
#87327=CARTESIAN_POINT('Ctrl Pts',(16.6845657868444,-19.4826219233898,-3.88069221239667));
#87328=CARTESIAN_POINT('Ctrl Pts',(16.6809624123329,-19.468508053008,-3.88155749452863));
#87329=CARTESIAN_POINT('Ctrl Pts',(16.6791671198924,-19.4613189002392,-3.88199643667253));
#87330=CARTESIAN_POINT('Ctrl Pts',(16.6747876940001,-19.4433815981793,-3.88308721527926));
#87331=CARTESIAN_POINT('Ctrl Pts',(16.6722499111464,-19.4326222780991,-3.88373756698111));
#87332=CARTESIAN_POINT('Ctrl Pts',(16.6345655722156,-19.2670604299227,-3.89368677446346));
#87333=CARTESIAN_POINT('Ctrl Pts',(16.6168549648591,-19.1088091393682,-3.90236291901907));
#87334=CARTESIAN_POINT('Ctrl Pts',(16.6170008943788,-18.9500540301098,-3.91098518891322));
#87335=CARTESIAN_POINT('Ctrl Pts',(16.6170008942721,-18.9500541461424,-3.91098518261129));
#87336=CARTESIAN_POINT('Ctrl Pts',(16.6171322450268,-18.807150592994,-3.91874652655734));
#87337=CARTESIAN_POINT('Ctrl Pts',(16.6317328278981,-18.6646421589114,-3.92644236870034));
#87338=CARTESIAN_POINT('Ctrl Pts',(16.6625397877042,-18.5151512563269,-3.93541346054193));
#87339=CARTESIAN_POINT('Ctrl Pts',(16.664575528335,-18.5056071413232,-3.93599028140181));
#87340=CARTESIAN_POINT('Ctrl Pts',(16.6678824993184,-18.4906120954945,-3.93690343976338));
#87341=CARTESIAN_POINT('Ctrl Pts',(16.6691095116038,-18.485151422396,-3.93723742441503));
#87342=CARTESIAN_POINT('Ctrl Pts',(16.6714748371374,-18.474816591108,-3.9378723699048));
#87343=CARTESIAN_POINT('Ctrl Pts',(16.6726088136726,-18.4699414673269,-3.93817308878256));
#87344=CARTESIAN_POINT('Ctrl Pts',(16.674595110385,-18.4615372783009,-3.93869364629781));
#87345=CARTESIAN_POINT('Ctrl Pts',(16.6754392482024,-18.458006263442,-3.93891301525651));
#87346=CARTESIAN_POINT('Ctrl Pts',(16.6770954348792,-18.451156427771,-3.93933987301878));
#87347=CARTESIAN_POINT('Ctrl Pts',(16.6779064366034,-18.4478373952451,-3.93954729529748));
#87348=CARTESIAN_POINT('Ctrl Pts',(16.6801203214834,-18.4388712398872,-3.94010920647488));
#87349=CARTESIAN_POINT('Ctrl Pts',(16.6815384461344,-18.4332279630271,-3.94046456097539));
#87350=CARTESIAN_POINT('Ctrl Pts',(16.6869129222515,-18.4122078196071,-3.9417943072034));
#87351=CARTESIAN_POINT('Ctrl Pts',(16.6910188485155,-18.396870211435,-3.94277680076158));
#87352=CARTESIAN_POINT('Ctrl Pts',(16.7288591366647,-18.2616273684232,-3.95153979924237));
#87353=CARTESIAN_POINT('Ctrl Pts',(16.7729395884032,-18.1448813410546,-3.9597852839377));
#87354=CARTESIAN_POINT('Ctrl Pts',(16.8579487258966,-17.9685399638464,-3.97272134811439));
#87355=CARTESIAN_POINT('Ctrl Pts',(16.8920974708809,-17.9059799623512,-3.97741803945359));
#87356=CARTESIAN_POINT('Ctrl Pts',(16.9785938462516,-17.7649381327066,-3.9881673007431));
#87357=CARTESIAN_POINT('Ctrl Pts',(17.0331635959518,-17.6879880280514,-3.99415312531795));
#87358=CARTESIAN_POINT('Ctrl Pts',(17.1062835262746,-17.5982306195257,-4.0012670795449));
#87359=CARTESIAN_POINT('Ctrl Pts',(17.1201345938356,-17.5817478484369,-4.00257972924413));
#87360=CARTESIAN_POINT('Ctrl Pts',(17.1388624500493,-17.5601396928721,-4.00430954043226));
#87361=CARTESIAN_POINT('Ctrl Pts',(17.1435165540233,-17.5548238021679,-4.00473583704547));
#87362=CARTESIAN_POINT('Ctrl Pts',(17.1527803127122,-17.5443490630269,-4.00557734893524));
#87363=CARTESIAN_POINT('Ctrl Pts',(17.1573888137821,-17.5391893159067,-4.00599260474899));
#87364=CARTESIAN_POINT('Ctrl Pts',(17.1663419748287,-17.5292635858118,-4.00679289665995));
#87365=CARTESIAN_POINT('Ctrl Pts',(17.1706832766093,-17.524494689352,-4.00717806750306));
#87366=CARTESIAN_POINT('Ctrl Pts',(17.1807335285554,-17.5135553773427,-4.00806318794605));
#87367=CARTESIAN_POINT('Ctrl Pts',(17.1864575991969,-17.5073989531388,-4.00856248736963));
#87368=CARTESIAN_POINT('Ctrl Pts',(17.2018963169743,-17.4909911835884,-4.00989648076564));
#87369=CARTESIAN_POINT('Ctrl Pts',(17.2116772341861,-17.4808025733234,-4.01072831994755));
#87370=CARTESIAN_POINT('Ctrl Pts',(17.2965477374868,-17.3941471641969,-4.01783566812774));
#87371=CARTESIAN_POINT('Ctrl Pts',(17.3772462405688,-17.3233815535954,-4.02384812440951));
#87372=CARTESIAN_POINT('Ctrl Pts',(17.5573816024749,-17.1881415195211,-4.03622324500037));
#87373=CARTESIAN_POINT('Ctrl Pts',(17.6575569873246,-17.125282499965,-4.0425373436808));
#87374=CARTESIAN_POINT('Ctrl Pts',(17.813994760785,-17.0444766133498,-4.05224394602577));
#87375=CARTESIAN_POINT('Ctrl Pts',(17.8666116221682,-17.0199825161489,-4.05548746685995));
#87376=CARTESIAN_POINT('Ctrl Pts',(17.9472478314773,-16.9864032006027,-4.06052050006638));
#87377=CARTESIAN_POINT('Ctrl Pts',(17.9745618845269,-16.9756894713332,-4.06223582584919));
#87378=CARTESIAN_POINT('Ctrl Pts',(18.008642825369,-16.9631322905427,-4.06439932129622));
#87379=CARTESIAN_POINT('Ctrl Pts',(18.0152093184098,-16.9607497019533,-4.06481722455301));
#87380=CARTESIAN_POINT('Ctrl Pts',(18.0256345172692,-16.9570253053494,-4.06548255138208));
#87381=CARTESIAN_POINT('Ctrl Pts',(18.0294855890195,-16.9556620693148,-4.06572872160866));
#87382=CARTESIAN_POINT('Ctrl Pts',(18.0367147507666,-16.9531265505232,-4.06619161649731));
#87383=CARTESIAN_POINT('Ctrl Pts',(18.0400918730844,-16.9519516764481,-4.06640818492256));
#87384=CARTESIAN_POINT('Ctrl Pts',(18.0478386314845,-16.94927862282,-4.06690570542153));
#87385=CARTESIAN_POINT('Ctrl Pts',(18.0522101929812,-16.9477861899567,-4.06718699230683));
#87386=CARTESIAN_POINT('Ctrl Pts',(18.0657708824511,-16.9432061279213,-4.06806111948406));
#87387=CARTESIAN_POINT('Ctrl Pts',(18.0749762081527,-16.940167350991,-4.06865672491701));
#87388=CARTESIAN_POINT('Ctrl Pts',(18.1796792826009,-16.9063994384453,-4.07545386053984));
#87389=CARTESIAN_POINT('Ctrl Pts',(18.2772139628935,-16.8824360721901,-4.08199312037277));
#87390=CARTESIAN_POINT('Ctrl Pts',(18.5450619534881,-16.836487907142,-4.09990016848115));
#87391=CARTESIAN_POINT('Ctrl Pts',(18.7169864911213,-16.8281313771881,-4.11128276028443));
#87392=CARTESIAN_POINT('Ctrl Pts',(18.9166113850612,-16.8426962769045,-4.12381584691051));
#87393=CARTESIAN_POINT('Ctrl Pts',(18.945128888553,-16.8453595867472,-4.12559196290256));
#87394=CARTESIAN_POINT('Ctrl Pts',(18.9941479474101,-16.8509430329236,-4.12862088491591));
#87395=CARTESIAN_POINT('Ctrl Pts',(19.0146762946979,-16.8535867426123,-4.12988205114767));
#87396=CARTESIAN_POINT('Ctrl Pts',(19.044069221094,-16.8578111273345,-4.13167787983704));
#87397=CARTESIAN_POINT('Ctrl Pts',(19.0529671349999,-16.8591478965386,-4.13222020963701));
#87398=CARTESIAN_POINT('Ctrl Pts',(19.0683017755664,-16.8615517497336,-4.13315267460102));
#87399=CARTESIAN_POINT('Ctrl Pts',(19.074742536386,-16.8625919284245,-4.13354365643846));
#87400=CARTESIAN_POINT('Ctrl Pts',(19.0870648929699,-16.8646404743521,-4.13429043610972));
#87401=CARTESIAN_POINT('Ctrl Pts',(19.0929472255147,-16.8656439665343,-4.13464638458562));
#87402=CARTESIAN_POINT('Ctrl Pts',(19.1082309880289,-16.8683178403119,-4.13556985788703));
#87403=CARTESIAN_POINT('Ctrl Pts',(19.1176255667072,-16.870026992463,-4.13613614588535));
#87404=CARTESIAN_POINT('Ctrl Pts',(19.1496143481711,-16.8760705734365,-4.13806001300611));
#87405=CARTESIAN_POINT('Ctrl Pts',(19.1721498128972,-16.8807098047414,-4.13940788880554));
#87406=CARTESIAN_POINT('Ctrl Pts',(19.3656821144205,-16.9238510634833,-4.15092960843955));
#87407=CARTESIAN_POINT('Ctrl Pts',(19.5313586195494,-16.9830824437085,-4.16035463219325));
#87408=CARTESIAN_POINT('Ctrl Pts',(19.7656511569744,-17.1013299881168,-4.17463384428289));
#87409=CARTESIAN_POINT('Ctrl Pts',(19.8409462725443,-17.1453591533735,-4.17940431541763));
#87410=CARTESIAN_POINT('Ctrl Pts',(19.9447486876472,-17.2149882134013,-4.18654043939971));
#87411=CARTESIAN_POINT('Ctrl Pts',(19.9756161257974,-17.2369165246796,-4.18873952418397));
#87412=CARTESIAN_POINT('Ctrl Pts',(20.0119313908688,-17.2642092184526,-4.19144234737294));
#87413=CARTESIAN_POINT('Ctrl Pts',(20.0179613398528,-17.2687918619851,-4.19189507126423));
#87414=CARTESIAN_POINT('Ctrl Pts',(20.0272829893438,-17.2759553691502,-4.19260129036553));
#87415=CARTESIAN_POINT('Ctrl Pts',(20.0305919199036,-17.2785138519628,-4.19285323308809));
#87416=CARTESIAN_POINT('Ctrl Pts',(20.0367060305067,-17.2832703339385,-4.19332113606196));
#87417=CARTESIAN_POINT('Ctrl Pts',(20.0395132508583,-17.285465616447,-4.19353690427466));
#87418=CARTESIAN_POINT('Ctrl Pts',(20.0458366172362,-17.2904363521236,-4.19402504293687));
#87419=CARTESIAN_POINT('Ctrl Pts',(20.0493494845876,-17.2932158673269,-4.1942977002401));
#87420=CARTESIAN_POINT('Ctrl Pts',(20.0596613368682,-17.3014283524415,-4.19510236547206));
#87421=CARTESIAN_POINT('Ctrl Pts',(20.0664355750082,-17.3068920472293,-4.19563650022051));
#87422=CARTESIAN_POINT('Ctrl Pts',(20.1142609018017,-17.3459542652007,-4.19944561028889));
#87423=CARTESIAN_POINT('Ctrl Pts',(20.1540666107663,-17.3810407836746,-4.20281658411742));
#87424=CARTESIAN_POINT('Ctrl Pts',(20.2031407328953,-17.4276871496822,-4.20719151568062));
#87425=CARTESIAN_POINT('Ctrl Pts',(20.2136669332617,-17.4379029387482,-4.20814353803682));
#87426=CARTESIAN_POINT('Ctrl Pts',(20.3360684427876,-17.559190381806,-4.21936749038897));
#87427=CARTESIAN_POINT('Ctrl Pts',(20.4353191157243,-17.6823298164806,-4.22994489757944));
#87428=CARTESIAN_POINT('Ctrl Pts',(20.5622276355565,-17.8817357765132,-4.24516587916816));
#87429=CARTESIAN_POINT('Ctrl Pts',(20.6007489992924,-17.950435009645,-4.25012587390771));
#87430=CARTESIAN_POINT('Ctrl Pts',(20.64384402799,-18.0384589932508,-4.25613296943187));
#87431=CARTESIAN_POINT('Ctrl Pts',(20.6520921023564,-18.0559061947288,-4.25730750637208));
#87432=CARTESIAN_POINT('Ctrl Pts',(20.6636877172089,-18.0813284048728,-4.25899618570591));
#87433=CARTESIAN_POINT('Ctrl Pts',(20.6672265924911,-18.0892145932762,-4.25951690101564));
#87434=CARTESIAN_POINT('Ctrl Pts',(20.6733270889082,-18.1030352089832,-4.26042407650483));
#87435=CARTESIAN_POINT('Ctrl Pts',(20.6759099976907,-18.1089600623545,-4.26081126257151));
#87436=CARTESIAN_POINT('Ctrl Pts',(20.6808588888161,-18.1204555962414,-4.26155920738928));
#87437=CARTESIAN_POINT('Ctrl Pts',(20.6832281931125,-18.1260247699052,-4.26192007655446));
#87438=CARTESIAN_POINT('Ctrl Pts',(20.6888135317041,-18.1393112807005,-4.26277752508377));
#87439=CARTESIAN_POINT('Ctrl Pts',(20.6920078119325,-18.14703769674,-4.26327336314781));
#87440=CARTESIAN_POINT('Ctrl Pts',(20.7032505681011,-18.1746949086611,-4.26503849117533));
#87441=CARTESIAN_POINT('Ctrl Pts',(20.7110413474744,-18.1947295295945,-4.26629910137887));
#87442=CARTESIAN_POINT('Ctrl Pts',(20.7851008758058,-18.394117725974,-4.27867745431361));
#87443=CARTESIAN_POINT('Ctrl Pts',(20.8270869071199,-18.5815407342442,-4.28887559396418));
#87444=CARTESIAN_POINT('Ctrl Pts',(20.8448918862198,-18.7902653813083,-4.3003100274299));
#87445=CARTESIAN_POINT('Ctrl Pts',(20.8462087670023,-18.8084843100314,-4.30130965431589));
#87446=CARTESIAN_POINT('Ctrl Pts',(20.8510070428199,-18.8894227599961,-4.3057654180126));
#87447=CARTESIAN_POINT('Ctrl Pts',(20.8519314225192,-18.9522576988149,-4.30926363796277));
#87448=CARTESIAN_POINT('Ctrl Pts',(20.849139428657,-19.0459828194259,-4.31465688290954));
#87449=CARTESIAN_POINT('Ctrl Pts',(20.847538809199,-19.0769041523292,-4.3164648639232));
#87450=CARTESIAN_POINT('Ctrl Pts',(20.8447361385059,-19.1148889285882,-4.31873321641045));
#87451=CARTESIAN_POINT('Ctrl Pts',(20.8441754997984,-19.1219976653006,-4.31915977826667));
#87452=CARTESIAN_POINT('Ctrl Pts',(20.8432371618529,-19.1331747455037,-4.31983387210236));
#87453=CARTESIAN_POINT('Ctrl Pts',(20.8428835749369,-19.1372451350554,-4.32008007080195));
#87454=CARTESIAN_POINT('Ctrl Pts',(20.8421984554848,-19.1448757567485,-4.32054298910724));
#87455=CARTESIAN_POINT('Ctrl Pts',(20.8418696855567,-19.148436181193,-4.32075955229524));
#87456=CARTESIAN_POINT('Ctrl Pts',(20.8410955761397,-19.1565936563274,-4.32125702064421));
#87457=CARTESIAN_POINT('Ctrl Pts',(20.8406442130522,-19.1611900807342,-4.32153826035543));
#87458=CARTESIAN_POINT('Ctrl Pts',(20.8391992657662,-19.1754254890373,-4.32241209810004));
#87459=CARTESIAN_POINT('Ctrl Pts',(20.8381545555891,-19.1850589962553,-4.32300745868872));
#87460=CARTESIAN_POINT('Ctrl Pts',(20.8252845760865,-19.2965869227376,-4.32994383226708));
#87461=CARTESIAN_POINT('Ctrl Pts',(20.8061357762546,-19.397488101707,-4.33663765486278));
#87462=CARTESIAN_POINT('Ctrl Pts',(20.750556775186,-19.6062705190626,-4.35088033031));
#87463=CARTESIAN_POINT('Ctrl Pts',(20.7125840652424,-19.7134323845532,-4.35841699205622));
#87464=CARTESIAN_POINT('Ctrl Pts',(20.6406403324251,-19.8741305395517,-4.36979857556154));
#87465=CARTESIAN_POINT('Ctrl Pts',(20.6125598904463,-19.9300674802251,-4.37377946027903));
#87466=CARTESIAN_POINT('Ctrl Pts',(20.5637103667782,-20.0174862935634,-4.38002097853965));
#87467=CARTESIAN_POINT('Ctrl Pts',(20.5445088835228,-20.0497973103322,-4.38233289887023));
#87468=CARTESIAN_POINT('Ctrl Pts',(20.5184970648319,-20.0910276398573,-4.38529152193148));
#87469=CARTESIAN_POINT('Ctrl Pts',(20.5124629895278,-20.1004263760125,-4.38596656429279));
#87470=CARTESIAN_POINT('Ctrl Pts',(20.5025388203374,-20.1156185479077,-4.38705881912149));
#87471=CARTESIAN_POINT('Ctrl Pts',(20.4986940244358,-20.1214411853572,-4.38747771179553));
#87472=CARTESIAN_POINT('Ctrl Pts',(20.491251790785,-20.1325915753133,-4.38828045549983));
#87473=CARTESIAN_POINT('Ctrl Pts',(20.4876587406391,-20.1379221503561,-4.38866446542979));
#87474=CARTESIAN_POINT('Ctrl Pts',(20.4793861792415,-20.1500753435945,-4.3895405862509));
#87475=CARTESIAN_POINT('Ctrl Pts',(20.4746908245431,-20.1568870901183,-4.3900320903874));
#87476=CARTESIAN_POINT('Ctrl Pts',(20.4621325456825,-20.1748792767801,-4.39133163607962));
#87477=CARTESIAN_POINT('Ctrl Pts',(20.4542009880882,-20.1860115050842,-4.39213705283293));
#87478=CARTESIAN_POINT('Ctrl Pts',(20.3943245239867,-20.2683510604055,-4.39810626087974));
#87479=CARTESIAN_POINT('Ctrl Pts',(20.3380825057733,-20.3363336483364,-4.40309658136059));
#87480=CARTESIAN_POINT('Ctrl Pts',(20.1816587004008,-20.5030309732924,-4.41576490590478));
#87481=CARTESIAN_POINT('Ctrl Pts',(20.0756097215768,-20.5956223510044,-4.42323448884659));
#87482=CARTESIAN_POINT('Ctrl Pts',(19.9153729328119,-20.709613924748,-4.43408921663631));
#87483=CARTESIAN_POINT('Ctrl Pts',(19.8682928023491,-20.7403589316955,-4.43723642182673));
#87484=CARTESIAN_POINT('Ctrl Pts',(19.7953303218629,-20.7839651186258,-4.44213758532606));
#87485=CARTESIAN_POINT('Ctrl Pts',(19.7703143354167,-20.7982314753511,-4.44382210296991));
#87486=CARTESIAN_POINT('Ctrl Pts',(19.7388943896497,-20.8153101785417,-4.44595269780006));
#87487=CARTESIAN_POINT('Ctrl Pts',(19.7327558788901,-20.8186076843058,-4.44636964464494));
#87488=CARTESIAN_POINT('Ctrl Pts',(19.72302427072,-20.8237735954388,-4.44703191632725));
#87489=CARTESIAN_POINT('Ctrl Pts',(19.7194418366185,-20.8256621324733,-4.44727598481943));
#87490=CARTESIAN_POINT('Ctrl Pts',(19.7126803309807,-20.8292018119008,-4.44773719199818));
#87491=CARTESIAN_POINT('Ctrl Pts',(19.7095024796353,-20.8308551685444,-4.44795418794132));
#87492=CARTESIAN_POINT('Ctrl Pts',(19.7022340422686,-20.8346133438917,-4.44845102228282));
#87493=CARTESIAN_POINT('Ctrl Pts',(19.698140787309,-20.8367128971099,-4.44873118703654));
#87494=CARTESIAN_POINT('Ctrl Pts',(19.6872693707117,-20.8422444893672,-4.44947620041015));
#87495=CARTESIAN_POINT('Ctrl Pts',(19.6804795925781,-20.8456533736611,-4.44994243968108));
#87496=CARTESIAN_POINT('Ctrl Pts',(19.6331949195803,-20.8690753406769,-4.45319511001396));
#87497=CARTESIAN_POINT('Ctrl Pts',(19.5920899380711,-20.8878229155986,-4.45605162024559));
#87498=CARTESIAN_POINT('Ctrl Pts',(19.5448560577405,-20.9075658581413,-4.45934132248214));
#87499=CARTESIAN_POINT('Ctrl Pts',(19.5392817973918,-20.9098678702855,-4.45972966979974));
#87500=CARTESIAN_POINT('Ctrl Pts',(19.387857283215,-20.9716458467912,-4.47028091976166));
#87501=CARTESIAN_POINT('Ctrl Pts',(19.2358317032477,-21.0146844976715,-4.48087241961921));
#87502=CARTESIAN_POINT('Ctrl Pts',(18.9788228692162,-21.0573169277316,-4.49778522002511));
#87503=CARTESIAN_POINT('Ctrl Pts',(18.8761075578689,-21.0667360381832,-4.50430455008965));
#87504=CARTESIAN_POINT('Ctrl Pts',(18.7582955273138,-21.0689123718683,-4.51149026778077));
#87505=CARTESIAN_POINT('Ctrl Pts',(18.743487780466,-21.0690305293784,-4.51238839611533));
#87506=CARTESIAN_POINT('Ctrl Pts',(18.7209110693839,-21.0689737910691,-4.51375029557122));
#87507=CARTESIAN_POINT('Ctrl Pts',(18.7131425145082,-21.0689115049965,-4.51421757808872));
#87508=CARTESIAN_POINT('Ctrl Pts',(18.6990135877202,-21.0687204393229,-4.51506505369275));
#87509=CARTESIAN_POINT('Ctrl Pts',(18.6926531456789,-21.0686057512671,-4.51544568343714));
#87510=CARTESIAN_POINT('Ctrl Pts',(18.678927497251,-21.0682963642911,-4.51626521193568));
#87511=CARTESIAN_POINT('Ctrl Pts',(18.6715625782903,-21.0680918818769,-4.51670379935123));
#87512=CARTESIAN_POINT('Ctrl Pts',(18.6516069289948,-21.0674335512477,-4.51788912828049));
#87513=CARTESIAN_POINT('Ctrl Pts',(18.6390188136284,-21.0669057455247,-4.51863354890142));
#87514=CARTESIAN_POINT('Ctrl Pts',(18.5779506916085,-21.0637988820969,-4.52222981640151));
#87515=CARTESIAN_POINT('Ctrl Pts',(18.5295622256888,-21.0596649717319,-4.52503268904232));
#87516=CARTESIAN_POINT('Ctrl Pts',(18.4408419156624,-21.0490008166845,-4.53011153237708));
#87517=CARTESIAN_POINT('Ctrl Pts',(18.4004759823562,-21.0429605598862,-4.53239921614737));
#87518=CARTESIAN_POINT('Ctrl Pts',(18.2279684054836,-21.0120238199983,-4.54212598747358));
#87519=CARTESIAN_POINT('Ctrl Pts',(18.0981946245966,-20.9757383575991,-4.5492958221996));
#87520=CARTESIAN_POINT('Ctrl Pts',(17.9142085627967,-20.9048352846544,-4.56013213438817));
#87521=CARTESIAN_POINT('Ctrl Pts',(17.8567131831197,-20.8796904162313,-4.56362568054111));
#87522=CARTESIAN_POINT('Ctrl Pts',(17.7726608082376,-20.8383914751444,-4.56901240883797));
#87523=CARTESIAN_POINT('Ctrl Pts',(17.7452021849488,-20.8241443568537,-4.57081879404963));
#87524=CARTESIAN_POINT('Ctrl Pts',(17.7118128666005,-20.8058806015747,-4.57308536833362));
#87525=CARTESIAN_POINT('Ctrl Pts',(17.7055759492039,-20.8024280015811,-4.57351181055268));
#87526=CARTESIAN_POINT('Ctrl Pts',(17.6957925308526,-20.7969474086559,-4.57418575733014));
#87527=CARTESIAN_POINT('Ctrl Pts',(17.6922341929193,-20.7949405015486,-4.57443192957794));
#87528=CARTESIAN_POINT('Ctrl Pts',(17.6855723074812,-20.7911577309575,-4.57489482612849));
#87529=CARTESIAN_POINT('Ctrl Pts',(17.6824674425733,-20.7893842999692,-4.57511139418157));
#87530=CARTESIAN_POINT('Ctrl Pts',(17.6753618234,-20.7853018160686,-4.57560891097636));
#87531=CARTESIAN_POINT('Ctrl Pts',(17.6713641352488,-20.7829875356665,-4.57589019451129));
#87532=CARTESIAN_POINT('Ctrl Pts',(17.6590006636788,-20.7757761363526,-4.57676430113089));
#87533=CARTESIAN_POINT('Ctrl Pts',(17.6506610564777,-20.7708347076815,-4.57735988917283));
#87534=CARTESIAN_POINT('Ctrl Pts',(17.5601865997406,-20.7163833160125,-4.58388409806534));
#87535=CARTESIAN_POINT('Ctrl Pts',(17.4814819645658,-20.6614094318154,-4.59012186014501));
#87536=CARTESIAN_POINT('Ctrl Pts',(17.3080639734281,-20.5218573464661,-4.60477487783295));
#87537=CARTESIAN_POINT('Ctrl Pts',(17.2166671805567,-20.4337055043317,-4.61320498130753));
#87538=CARTESIAN_POINT('Ctrl Pts',(17.095548957908,-20.2938507932039,-4.62512680015848));
#87539=CARTESIAN_POINT('Ctrl Pts',(17.0592296961152,-20.2482371535256,-4.62882514592249));
#87540=CARTESIAN_POINT('Ctrl Pts',(17.003757511288,-20.1723384975902,-4.63467551855821));
#87541=CARTESIAN_POINT('Ctrl Pts',(16.9834109851594,-20.1429674486201,-4.63687122488612));
#87542=CARTESIAN_POINT('Ctrl Pts',(16.9578007277931,-20.1039225028554,-4.63970427586288));
#87543=CARTESIAN_POINT('Ctrl Pts',(16.9518562258008,-20.0947041972219,-4.6403670700672));
#87544=CARTESIAN_POINT('Ctrl Pts',(16.942271512775,-20.0795841864198,-4.64144445219298));
#87545=CARTESIAN_POINT('Ctrl Pts',(16.938588233542,-20.073710149745,-4.64186063588693));
#87546=CARTESIAN_POINT('Ctrl Pts',(16.9315377479591,-20.0623424453259,-4.64266153176346));
#87547=CARTESIAN_POINT('Ctrl Pts',(16.9281666400029,-20.0568512991635,-4.64304638494522));
#87548=CARTESIAN_POINT('Ctrl Pts',(16.9204737008798,-20.0441911157656,-4.64392910686645));
#87549=CARTESIAN_POINT('Ctrl Pts',(16.9161691975441,-20.0370116348093,-4.64442633698628));
#87550=CARTESIAN_POINT('Ctrl Pts',(16.9047787872845,-20.0177555081973,-4.64575115690543));
#87551=CARTESIAN_POINT('Ctrl Pts',(16.8977698422501,-20.005633650806,-4.64657595408827));
#87552=CARTESIAN_POINT('Ctrl Pts',(16.8410108978301,-19.9051831555845,-4.65333769699532));
#87553=CARTESIAN_POINT('Ctrl Pts',(16.7975407853625,-19.8134495866659,-4.65904106758851));
#87554=CARTESIAN_POINT('Ctrl Pts',(16.7555370085584,-19.7053822958017,-4.66542624492597));
#87555=CARTESIAN_POINT('Ctrl Pts',(16.7504072892657,-19.6917705270986,-4.66622485003499));
#87556=CARTESIAN_POINT('Ctrl Pts',(16.7454194642264,-19.6781104962347,-4.66702132639115));
#87557=CARTESIAN_POINT('',(16.6170000029932,-18.9521080403316,-3.68920542528284));
#87558=CARTESIAN_POINT('Ctrl Pts',(16.7454194481082,-19.6781104520924,-4.44630497675564));
#87559=CARTESIAN_POINT('Ctrl Pts',(16.7620249650105,-19.7235875663122,-4.44325057402068));
#87560=CARTESIAN_POINT('Ctrl Pts',(16.7801860421437,-19.7684827781901,-4.44012924995249));
#87561=CARTESIAN_POINT('Ctrl Pts',(16.8760920334208,-19.9839946047985,-4.42474708274802));
#87562=CARTESIAN_POINT('Ctrl Pts',(16.9747456752738,-20.1444254883296,-4.41214842939464));
#87563=CARTESIAN_POINT('Ctrl Pts',(17.128653912656,-20.3331925216919,-4.39674509008298));
#87564=CARTESIAN_POINT('Ctrl Pts',(17.1657754045437,-20.375201105423,-4.39326452551378));
#87565=CARTESIAN_POINT('Ctrl Pts',(17.21284242246,-20.4243835799468,-4.38912058938185));
#87566=CARTESIAN_POINT('Ctrl Pts',(17.2212358015587,-20.4330058310142,-4.38839135267341));
#87567=CARTESIAN_POINT('Ctrl Pts',(17.235236630318,-20.4471452193277,-4.38719075166915));
#87568=CARTESIAN_POINT('Ctrl Pts',(17.2408020475568,-20.4527034159365,-4.38671755806291));
#87569=CARTESIAN_POINT('Ctrl Pts',(17.2509287309101,-20.4627048535588,-4.3858637855344));
#87570=CARTESIAN_POINT('Ctrl Pts',(17.2554792912079,-20.4671587569661,-4.38548273811394));
#87571=CARTESIAN_POINT('Ctrl Pts',(17.2652853251112,-20.4766702597563,-4.38466714512043));
#87572=CARTESIAN_POINT('Ctrl Pts',(17.2705469922286,-20.4817213776718,-4.38423288508739));
#87573=CARTESIAN_POINT('Ctrl Pts',(17.2849676767021,-20.4954225059504,-4.38305175830486));
#87574=CARTESIAN_POINT('Ctrl Pts',(17.2941780608875,-20.5040182021533,-4.38230723643732));
#87575=CARTESIAN_POINT('Ctrl Pts',(17.3433130876007,-20.5490601604775,-4.37838616728606));
#87576=CARTESIAN_POINT('Ctrl Pts',(17.3845480436711,-20.5840512815691,-4.37527146400633));
#87577=CARTESIAN_POINT('Ctrl Pts',(17.5775416422962,-20.7355001608935,-4.36137520466466));
#87578=CARTESIAN_POINT('Ctrl Pts',(17.7432941334274,-20.832628873766,-4.35135116592928));
#87579=CARTESIAN_POINT('Ctrl Pts',(17.9351027651706,-20.9125422710085,-4.33980018923013));
#87580=CARTESIAN_POINT('Ctrl Pts',(17.9504505020504,-20.918726455928,-4.33887558096187));
#87581=CARTESIAN_POINT('Ctrl Pts',(18.0154338884566,-20.9440293422559,-4.33495322844088));
#87582=CARTESIAN_POINT('Ctrl Pts',(18.0657043284998,-20.9614521744423,-4.33190078574014));
#87583=CARTESIAN_POINT('Ctrl Pts',(18.1249045864624,-20.9795028121471,-4.32822792058208));
#87584=CARTESIAN_POINT('Ctrl Pts',(18.1332520097391,-20.9819918035192,-4.32770824988559));
#87585=CARTESIAN_POINT('Ctrl Pts',(18.145916551802,-20.985683096966,-4.32691678488499));
#87586=CARTESIAN_POINT('Ctrl Pts',(18.150222636011,-20.9869233571255,-4.32664714925575));
#87587=CARTESIAN_POINT('Ctrl Pts',(18.1579603156129,-20.9891254215144,-4.32616163403157));
#87588=CARTESIAN_POINT('Ctrl Pts',(18.1613904278957,-20.9900922399649,-4.3259460498309));
#87589=CARTESIAN_POINT('Ctrl Pts',(18.1688504954415,-20.9921746302837,-4.32547639755785));
#87590=CARTESIAN_POINT('Ctrl Pts',(18.1728812667483,-20.993286910518,-4.32522214765856));
#87591=CARTESIAN_POINT('Ctrl Pts',(18.1842164922373,-20.9963787243408,-4.32450582769488));
#87592=CARTESIAN_POINT('Ctrl Pts',(18.1915282185601,-20.9983310182653,-4.32404222560675));
#87593=CARTESIAN_POINT('Ctrl Pts',(18.2353814012106,-21.0097886496481,-4.32125312558855));
#87594=CARTESIAN_POINT('Ctrl Pts',(18.2721589538434,-21.0183535694137,-4.31887852524716));
#87595=CARTESIAN_POINT('Ctrl Pts',(18.3941219554129,-21.0433384188235,-4.31093049535583));
#87596=CARTESIAN_POINT('Ctrl Pts',(18.480085226604,-21.055506321663,-4.30521499128242));
#87597=CARTESIAN_POINT('Ctrl Pts',(18.7418155003558,-21.0762741531225,-4.28786816794678));
#87598=CARTESIAN_POINT('Ctrl Pts',(18.9181715414562,-21.0682953942103,-4.27632337986769));
#87599=CARTESIAN_POINT('Ctrl Pts',(19.1141662730203,-21.0347121598167,-4.26408405468157));
#87600=CARTESIAN_POINT('Ctrl Pts',(19.1367362652717,-21.0304657566607,-4.26268221875535));
#87601=CARTESIAN_POINT('Ctrl Pts',(19.1685805919242,-21.0239362326402,-4.26071444128344));
#87602=CARTESIAN_POINT('Ctrl Pts',(19.1779148194114,-21.0219564441732,-4.26013887635612));
#87603=CARTESIAN_POINT('Ctrl Pts',(19.1930631187195,-21.0186363119889,-4.25920672641979));
#87604=CARTESIAN_POINT('Ctrl Pts',(19.1988853939554,-21.0173343953508,-4.25884891550203));
#87605=CARTESIAN_POINT('Ctrl Pts',(19.2110640127712,-21.014557031007,-4.25810141160334));
#87606=CARTESIAN_POINT('Ctrl Pts',(19.2174192032255,-21.0130767704918,-4.25771187754814));
#87607=CARTESIAN_POINT('Ctrl Pts',(19.2325268295404,-21.0094841590691,-4.25678710379233));
#87608=CARTESIAN_POINT('Ctrl Pts',(19.2412728790618,-21.0073452981371,-4.25625272323438));
#87609=CARTESIAN_POINT('Ctrl Pts',(19.2707159145857,-20.999945569871,-4.25445688936834));
#87610=CARTESIAN_POINT('Ctrl Pts',(19.2913472933398,-20.9944272505649,-4.2532037472672));
#87611=CARTESIAN_POINT('Ctrl Pts',(19.4033611442526,-20.9626428990166,-4.24642344098933));
#87612=CARTESIAN_POINT('Ctrl Pts',(19.4929832452532,-20.9305541927143,-4.24109059784727));
#87613=CARTESIAN_POINT('Ctrl Pts',(19.7363294033509,-20.8244458185074,-4.22648539037809));
#87614=CARTESIAN_POINT('Ctrl Pts',(19.8836950237315,-20.7377511031314,-4.21752245334345));
#87615=CARTESIAN_POINT('Ctrl Pts',(20.0485720538876,-20.6118096533522,-4.20567638964912));
#87616=CARTESIAN_POINT('Ctrl Pts',(20.0774800446018,-20.5884989347384,-4.20352008597582));
#87617=CARTESIAN_POINT('Ctrl Pts',(20.1112138538258,-20.559800456601,-4.20088710488825));
#87618=CARTESIAN_POINT('Ctrl Pts',(20.1166459097343,-20.5551314956709,-4.20045940006467));
#87619=CARTESIAN_POINT('Ctrl Pts',(20.1254659567804,-20.5474723157477,-4.19975863629244));
#87620=CARTESIAN_POINT('Ctrl Pts',(20.1288683033351,-20.5444986137129,-4.19948677182063));
#87621=CARTESIAN_POINT('Ctrl Pts',(20.1349389239234,-20.5391584204026,-4.1989988741905));
#87622=CARTESIAN_POINT('Ctrl Pts',(20.1376107612441,-20.5367960596454,-4.19878314911413));
#87623=CARTESIAN_POINT('Ctrl Pts',(20.1433811896968,-20.5316679752768,-4.19831508456265));
#87624=CARTESIAN_POINT('Ctrl Pts',(20.1464775726212,-20.5288999195079,-4.19806257353658));
#87625=CARTESIAN_POINT('Ctrl Pts',(20.1550968878815,-20.5211488040496,-4.19735593901223));
#87626=CARTESIAN_POINT('Ctrl Pts',(20.1606016680782,-20.5161457767283,-4.1969003479617));
#87627=CARTESIAN_POINT('Ctrl Pts',(20.1922825458036,-20.487046205167,-4.19425399916898));
#87628=CARTESIAN_POINT('Ctrl Pts',(20.2178725897038,-20.4623233518713,-4.19201969066369));
#87629=CARTESIAN_POINT('Ctrl Pts',(20.2978747302283,-20.3810359527808,-4.18475220594539));
#87630=CARTESIAN_POINT('Ctrl Pts',(20.3497672864184,-20.322088442459,-4.17960070547353));
#87631=CARTESIAN_POINT('Ctrl Pts',(20.5145165245978,-20.1125302008044,-4.16200627179355));
#87632=CARTESIAN_POINT('Ctrl Pts',(20.6105698709585,-19.9497894169119,-4.14960150739656));
#87633=CARTESIAN_POINT('Ctrl Pts',(20.6923612119241,-19.7563553017386,-4.13668939720248));
#87634=CARTESIAN_POINT('Ctrl Pts',(20.7005561660786,-19.7361064912185,-4.13535699814116));
#87635=CARTESIAN_POINT('Ctrl Pts',(20.7114730724325,-19.7078836512959,-4.13352579551715));
#87636=CARTESIAN_POINT('Ctrl Pts',(20.7144628107774,-19.7000153105525,-4.13301802458144));
#87637=CARTESIAN_POINT('Ctrl Pts',(20.7195266532424,-19.6864451763178,-4.1321469695101));
#87638=CARTESIAN_POINT('Ctrl Pts',(20.7216233026992,-19.6807519574665,-4.13178293402681));
#87639=CARTESIAN_POINT('Ctrl Pts',(20.7259001015553,-19.6689830201237,-4.13103327451251));
#87640=CARTESIAN_POINT('Ctrl Pts',(20.7280769970745,-19.6629061800859,-4.1306477621981));
#87641=CARTESIAN_POINT('Ctrl Pts',(20.7330862708609,-19.6487186554223,-4.12975132131604));
#87642=CARTESIAN_POINT('Ctrl Pts',(20.7358971533161,-19.6406004603696,-4.12924111098228));
#87643=CARTESIAN_POINT('Ctrl Pts',(20.7447679816001,-19.6144668980911,-4.1276072886998));
#87644=CARTESIAN_POINT('Ctrl Pts',(20.7506348627138,-19.5963866325681,-4.12649005023018));
#87645=CARTESIAN_POINT('Ctrl Pts',(20.7788916609616,-19.5051380761807,-4.12091372228174));
#87646=CARTESIAN_POINT('Ctrl Pts',(20.7975478867688,-19.4308690300516,-4.1165776338642));
#87647=CARTESIAN_POINT('Ctrl Pts',(20.8330979413149,-19.2478875854949,-4.10621827960241));
#87648=CARTESIAN_POINT('Ctrl Pts',(20.8456243471935,-19.1385611644657,-4.10030441919368));
#87649=CARTESIAN_POINT('Ctrl Pts',(20.8521447173799,-18.9588373472105,-4.09050992506386));
#87650=CARTESIAN_POINT('Ctrl Pts',(20.851213659677,-18.8888416956147,-4.08667438613998));
#87651=CARTESIAN_POINT('Ctrl Pts',(20.8437800173909,-18.7707295118865,-4.079990300364));
#87652=CARTESIAN_POINT('Ctrl Pts',(20.8390856216013,-18.7225562039939,-4.0772036432575));
#87653=CARTESIAN_POINT('Ctrl Pts',(20.8317297155465,-18.6669050425509,-4.07387092628283));
#87654=CARTESIAN_POINT('Ctrl Pts',(20.8306717068757,-18.6592256095969,-4.07340851279436));
#87655=CARTESIAN_POINT('Ctrl Pts',(20.8289122270146,-18.6469535373236,-4.07266526833124));
#87656=CARTESIAN_POINT('Ctrl Pts',(20.8282377618997,-18.6423570136777,-4.07238592133023));
#87657=CARTESIAN_POINT('Ctrl Pts',(20.8270155818869,-18.6342144617413,-4.07188930190836));
#87658=CARTESIAN_POINT('Ctrl Pts',(20.8264739755968,-18.6306675621209,-4.07167237738703));
#87659=CARTESIAN_POINT('Ctrl Pts',(20.8253059220791,-18.6231463435563,-4.07121110022692));
#87660=CARTESIAN_POINT('Ctrl Pts',(20.8246771715133,-18.6191724906672,-4.07096662488864));
#87661=CARTESIAN_POINT('Ctrl Pts',(20.8229474752499,-18.6084387179358,-4.07030426686697));
#87662=CARTESIAN_POINT('Ctrl Pts',(20.8218250570873,-18.6016823770901,-4.06988519565038));
#87663=CARTESIAN_POINT('Ctrl Pts',(20.8160626691347,-18.5680075822169,-4.06778613343214));
#87664=CARTESIAN_POINT('Ctrl Pts',(20.8109350256201,-18.5411765947512,-4.06608069682155));
#87665=CARTESIAN_POINT('Ctrl Pts',(20.7945570946609,-18.4636454696931,-4.06107120426277));
#87666=CARTESIAN_POINT('Ctrl Pts',(20.7819589992993,-18.4132524724586,-4.05771361070909));
#87667=CARTESIAN_POINT('Ctrl Pts',(20.7289403618539,-18.2300883454846,-4.04524807277243));
#87668=CARTESIAN_POINT('Ctrl Pts',(20.6773432552504,-18.1009038521253,-4.03596899587365));
#87669=CARTESIAN_POINT('Ctrl Pts',(20.569549357182,-17.8929641326548,-4.02080822720532));
#87670=CARTESIAN_POINT('Ctrl Pts',(20.519939416656,-17.8112882985431,-4.01478011230963));
#87671=CARTESIAN_POINT('Ctrl Pts',(20.4570007153589,-17.7218985473351,-4.00810853364584));
#87672=CARTESIAN_POINT('Ctrl Pts',(20.448911262178,-17.7106457289853,-4.00726709431055));
#87673=CARTESIAN_POINT('Ctrl Pts',(20.4357839605596,-17.6927582752486,-4.00592677553272));
#87674=CARTESIAN_POINT('Ctrl Pts',(20.4308165426145,-17.686072674448,-4.00542518911778));
#87675=CARTESIAN_POINT('Ctrl Pts',(20.4219404330924,-17.6742725148358,-4.00453869918699));
#87676=CARTESIAN_POINT('Ctrl Pts',(20.4180476507871,-17.6691461722745,-4.00415318056397));
#87677=CARTESIAN_POINT('Ctrl Pts',(20.4099021345018,-17.6585204437411,-4.00335321393102));
#87678=CARTESIAN_POINT('Ctrl Pts',(20.4056455660315,-17.6530240840469,-4.00293892353501));
#87679=CARTESIAN_POINT('Ctrl Pts',(20.394551602368,-17.6388436745648,-4.00186872197426));
#87680=CARTESIAN_POINT('Ctrl Pts',(20.3876730806668,-17.630191954767,-4.00121445382104));
#87681=CARTESIAN_POINT('Ctrl Pts',(20.3577945671135,-17.5932094325945,-3.99841151329896));
#87682=CARTESIAN_POINT('Ctrl Pts',(20.3341311157104,-17.5654210264271,-3.9962897026237));
#87683=CARTESIAN_POINT('Ctrl Pts',(20.2696696035534,-17.4935721330939,-3.99074664840355));
#87684=CARTESIAN_POINT('Ctrl Pts',(20.2276947671477,-17.4506107377091,-3.98737330512819));
#87685=CARTESIAN_POINT('Ctrl Pts',(20.0623019353966,-17.2951427957841,-3.97479978143302));
#87686=CARTESIAN_POINT('Ctrl Pts',(19.9275687119945,-17.1955979680647,-3.96600993986647));
#87687=CARTESIAN_POINT('Ctrl Pts',(19.7353207702023,-17.0859877027177,-3.95357489166082));
#87688=CARTESIAN_POINT('Ctrl Pts',(19.6870720111133,-17.0608897845281,-3.95045730470458));
#87689=CARTESIAN_POINT('Ctrl Pts',(19.6299947532243,-17.0339387053974,-3.94671185286621));
#87690=CARTESIAN_POINT('Ctrl Pts',(19.6220509553461,-17.0302478769698,-3.94618931103442));
#87691=CARTESIAN_POINT('Ctrl Pts',(19.609999507613,-17.0247392398269,-3.94539432409029));
#87692=CARTESIAN_POINT('Ctrl Pts',(19.6059084887512,-17.0228849797303,-3.94512406649636));
#87693=CARTESIAN_POINT('Ctrl Pts',(19.5985603566445,-17.0195825772687,-3.94463788927883));
#87694=CARTESIAN_POINT('Ctrl Pts',(19.5953054615797,-17.0181296301149,-3.94442226859365));
#87695=CARTESIAN_POINT('Ctrl Pts',(19.5882316074162,-17.0149933457851,-3.94395307218101));
#87696=CARTESIAN_POINT('Ctrl Pts',(19.5844113861944,-17.0133131013187,-3.94369931754476));
#87697=CARTESIAN_POINT('Ctrl Pts',(19.5736835928425,-17.0086325152324,-3.94298576058678));
#87698=CARTESIAN_POINT('Ctrl Pts',(19.5667650228792,-17.0056577562786,-3.94252444476115));
#87699=CARTESIAN_POINT('Ctrl Pts',(19.5256520504304,-16.9882398576705,-3.93977708139106));
#87700=CARTESIAN_POINT('Ctrl Pts',(19.4911006580505,-16.9746621254663,-3.93744359018556));
#87701=CARTESIAN_POINT('Ctrl Pts',(19.3770088902704,-16.9332558136414,-3.92969917909186));
#87702=CARTESIAN_POINT('Ctrl Pts',(19.2961644863234,-16.9092670826731,-3.92415347546493));
#87703=CARTESIAN_POINT('Ctrl Pts',(19.0393710327426,-16.8494711556924,-3.90673697666808));
#87704=CARTESIAN_POINT('Ctrl Pts',(18.8601281991922,-16.8311521249555,-3.894940877039));
#87705=CARTESIAN_POINT('Ctrl Pts',(18.6580305910556,-16.836242012828,-3.88250129712701));
#87706=CARTESIAN_POINT('Ctrl Pts',(18.6353715300587,-16.8371771471193,-3.88111727139148));
#87707=CARTESIAN_POINT('Ctrl Pts',(18.6032524350829,-16.8390200625245,-3.87916992712946));
#87708=CARTESIAN_POINT('Ctrl Pts',(18.5937773638064,-16.8396276940846,-3.87859725428967));
#87709=CARTESIAN_POINT('Ctrl Pts',(18.5783640516092,-16.8407203068642,-3.87766850697028));
#87710=CARTESIAN_POINT('Ctrl Pts',(18.5724232827596,-16.8411666440355,-3.87731122428192));
#87711=CARTESIAN_POINT('Ctrl Pts',(18.5599720562675,-16.8421549931263,-3.87656380481841));
#87712=CARTESIAN_POINT('Ctrl Pts',(18.553462055257,-16.8427020764688,-3.87617383144571));
#87713=CARTESIAN_POINT('Ctrl Pts',(18.5379446023199,-16.8440784880761,-3.87524615496126));
#87714=CARTESIAN_POINT('Ctrl Pts',(18.5289396809375,-16.8449354331668,-3.87470932552772));
#87715=CARTESIAN_POINT('Ctrl Pts',(18.4984479531313,-16.8480344748612,-3.87289646801807));
#87716=CARTESIAN_POINT('Ctrl Pts',(18.4769896258437,-16.8505477839949,-3.87162897072507));
#87717=CARTESIAN_POINT('Ctrl Pts',(18.4259255110994,-16.8573225665961,-3.86863011270599));
#87718=CARTESIAN_POINT('Ctrl Pts',(18.3963638303689,-16.8618838834215,-3.86690807199501));
#87719=CARTESIAN_POINT('Ctrl Pts',(18.1995919624353,-16.8965293882015,-3.85551679721451));
#87720=CARTESIAN_POINT('Ctrl Pts',(18.0364365937917,-16.9460193165672,-3.84647866167954));
#87721=CARTESIAN_POINT('Ctrl Pts',(17.7897507366714,-17.0546305161837,-3.83172673165066));
#87722=CARTESIAN_POINT('Ctrl Pts',(17.7015159568439,-17.1011653010719,-3.82618577307012));
#87723=CARTESIAN_POINT('Ctrl Pts',(17.608846029193,-17.1587327608825,-3.81972237605751));
#87724=CARTESIAN_POINT('Ctrl Pts',(17.6008281332082,-17.1637885019697,-3.81915758100142));
#87725=CARTESIAN_POINT('Ctrl Pts',(17.5889725964014,-17.1713758458612,-3.81831372157468));
#87726=CARTESIAN_POINT('Ctrl Pts',(17.5851086877815,-17.1738664602762,-3.81803730486337));
#87727=CARTESIAN_POINT('Ctrl Pts',(17.578316151441,-17.178276204665,-3.81754886996845));
#87728=CARTESIAN_POINT('Ctrl Pts',(17.575384133208,-17.1801900403714,-3.81733720612231));
#87729=CARTESIAN_POINT('Ctrl Pts',(17.5724288914134,-17.1821295073329,-3.81712301687775));
#87730=CARTESIAN_POINT('Ctrl Pts',(17.5724009498372,-17.1821478457854,-3.81712099165907));
#87731=CARTESIAN_POINT('Ctrl Pts',(17.5723459289161,-17.1821839586603,-3.81711700356618));
#87732=CARTESIAN_POINT('Ctrl Pts',(17.5723188494479,-17.182201733106,-3.81711504068768));
#87733=CARTESIAN_POINT('Ctrl Pts',(17.5722654881884,-17.1822367601698,-3.81711117260956));
#87734=CARTESIAN_POINT('Ctrl Pts',(17.5722392061731,-17.1822540128834,-3.81710926739788));
#87735=CARTESIAN_POINT('Ctrl Pts',(17.5721873807932,-17.1822880350787,-3.8171055103868));
#87736=CARTESIAN_POINT('Ctrl Pts',(17.572161837702,-17.1823048043344,-3.81710365861098));
#87737=CARTESIAN_POINT('Ctrl Pts',(17.5721114379439,-17.1823378937641,-3.81710000469647));
#87738=CARTESIAN_POINT('Ctrl Pts',(17.5720865812556,-17.1823542139101,-3.81709820255963));
#87739=CARTESIAN_POINT('Ctrl Pts',(17.5720375071393,-17.1823864359629,-3.81709464451364));
#87740=CARTESIAN_POINT('Ctrl Pts',(17.5720132894813,-17.1824023379826,-3.8170928885909));
#87741=CARTESIAN_POINT('Ctrl Pts',(17.5719654496359,-17.1824337524244,-3.81708941980716));
#87742=CARTESIAN_POINT('Ctrl Pts',(17.5719418276003,-17.1824492647122,-3.81708770695996));
#87743=CARTESIAN_POINT('Ctrl Pts',(17.5718951398951,-17.1824799252673,-3.81708432150007));
#87744=CARTESIAN_POINT('Ctrl Pts',(17.5718720741621,-17.1824950735448,-3.81708264888532));
#87745=CARTESIAN_POINT('Ctrl Pts',(17.5718264632201,-17.1825250295254,-3.81707934129875));
#87746=CARTESIAN_POINT('Ctrl Pts',(17.5718039178955,-17.1825398372756,-3.81707770632088));
#87747=CARTESIAN_POINT('Ctrl Pts',(17.5717593143917,-17.1825691340396,-3.81707447159432));
#87748=CARTESIAN_POINT('Ctrl Pts',(17.5717372563277,-17.1825836229514,-3.81707287185612));
#87749=CARTESIAN_POINT('Ctrl Pts',(17.571693597412,-17.1826123016221,-3.81706970544434));
#87750=CARTESIAN_POINT('Ctrl Pts',(17.5716719964266,-17.1826264914448,-3.81706813876303));
#87751=CARTESIAN_POINT('Ctrl Pts',(17.5716292235413,-17.1826545903424,-3.8170650364308));
#87752=CARTESIAN_POINT('Ctrl Pts',(17.5716080516702,-17.1826684993761,-3.81706350078379));
#87753=CARTESIAN_POINT('Ctrl Pts',(17.5715661111001,-17.1826960536543,-3.81706045864593));
#87754=CARTESIAN_POINT('Ctrl Pts',(17.5715453425134,-17.1827096988043,-3.81705895216489));
#87755=CARTESIAN_POINT('Ctrl Pts',(17.5715041845188,-17.1827367410179,-3.81705596662349));
#87756=CARTESIAN_POINT('Ctrl Pts',(17.5714837952355,-17.1827501379807,-3.81705448757369));
#87757=CARTESIAN_POINT('Ctrl Pts',(17.5714433739743,-17.1827766981361,-3.81705155531261));
#87758=CARTESIAN_POINT('Ctrl Pts',(17.5714233418685,-17.1827898613951,-3.81705010209346));
#87759=CARTESIAN_POINT('Ctrl Pts',(17.5713836146902,-17.182815967412,-3.8170472200272));
#87760=CARTESIAN_POINT('Ctrl Pts',(17.5713639193692,-17.1828289103168,-3.81704579116339));
#87761=CARTESIAN_POINT('Ctrl Pts',(17.5713248456554,-17.1828545887894,-3.81704295635311));
#87762=CARTESIAN_POINT('Ctrl Pts',(17.5713054675604,-17.1828673241465,-3.81704155042945));
#87763=CARTESIAN_POINT('Ctrl Pts',(17.5712670110983,-17.182892598783,-3.81703876025517));
#87764=CARTESIAN_POINT('Ctrl Pts',(17.5712479325239,-17.1829051381847,-3.81703737599063));
#87765=CARTESIAN_POINT('Ctrl Pts',(17.571210058131,-17.1829300320241,-3.81703462790649));
#87766=CARTESIAN_POINT('Ctrl Pts',(17.571191262281,-17.1829423864695,-3.81703326408565));
#87767=CARTESIAN_POINT('Ctrl Pts',(17.5711539374934,-17.1829669207715,-3.81703055574244));
#87768=CARTESIAN_POINT('Ctrl Pts',(17.5711354086296,-17.1829791005676,-3.81702921122638));
#87769=CARTESIAN_POINT('Ctrl Pts',(17.5710986029691,-17.1830032952937,-3.81702654041839));
#87770=CARTESIAN_POINT('Ctrl Pts',(17.571080326287,-17.183015310137,-3.81702521413569));
#87771=CARTESIAN_POINT('Ctrl Pts',(17.5710440112129,-17.1830391839811,-3.81702257879733));
#87772=CARTESIAN_POINT('Ctrl Pts',(17.5710259728216,-17.1830510429709,-3.81702126974257));
#87773=CARTESIAN_POINT('Ctrl Pts',(17.5709901215587,-17.1830746134723,-3.81701866793588));
#87774=CARTESIAN_POINT('Ctrl Pts',(17.5709723085161,-17.1830863250864,-3.81701737517233));
#87775=CARTESIAN_POINT('Ctrl Pts',(17.5709368953272,-17.1831096091073,-3.81701480503424));
#87776=CARTESIAN_POINT('Ctrl Pts',(17.5709192952055,-17.1831211814885,-3.81701352766225));
#87777=CARTESIAN_POINT('Ctrl Pts',(17.5708842964279,-17.1831441945321,-3.81701098747986));
#87778=CARTESIAN_POINT('Ctrl Pts',(17.5708668976816,-17.1831556352452,-3.81700972466362));
#87779=CARTESIAN_POINT('Ctrl Pts',(17.5708322903486,-17.1831783923616,-3.81700721277418));
#87780=CARTESIAN_POINT('Ctrl Pts',(17.5708150818517,-17.1831897086978,-3.81700596370815));
#87781=CARTESIAN_POINT('Ctrl Pts',(17.5707808447363,-17.1832122237976,-3.81700347857482));
#87782=CARTESIAN_POINT('Ctrl Pts',(17.5707638160636,-17.1832234225894,-3.81700224250417));
#87783=CARTESIAN_POINT('Ctrl Pts',(17.5707299289429,-17.1832457089267,-3.81699978266266));
#87784=CARTESIAN_POINT('Ctrl Pts',(17.570713070344,-17.1832567965647,-3.81699855888138));
#87785=CARTESIAN_POINT('Ctrl Pts',(17.5706795133068,-17.1832788671927,-3.81699612288973));
#87786=CARTESIAN_POINT('Ctrl Pts',(17.5706628150943,-17.1832898500277,-3.81699491069625));
#87787=CARTESIAN_POINT('Ctrl Pts',(17.5706295705404,-17.1833117164827,-3.81699249727998));
#87788=CARTESIAN_POINT('Ctrl Pts',(17.5706130239909,-17.1833226002335,-3.81699129604257));
#87789=CARTESIAN_POINT('Ctrl Pts',(17.5705800738538,-17.1833442743622,-3.81698890389308));
#87790=CARTESIAN_POINT('Ctrl Pts',(17.5705636703381,-17.183355064687,-3.81698771298669));
#87791=CARTESIAN_POINT('Ctrl Pts',(17.5705309980389,-17.1833765573602,-3.81698534090316));
#87792=CARTESIAN_POINT('Ctrl Pts',(17.5705147293416,-17.1833872596467,-3.81698415973269));
#87793=CARTESIAN_POINT('Ctrl Pts',(17.5704823191981,-17.1834085811487,-3.81698180657913));
#87794=CARTESIAN_POINT('Ctrl Pts',(17.5704661776557,-17.1834192004225,-3.81698063458944));
#87795=CARTESIAN_POINT('Ctrl Pts',(17.5669362988661,-17.1857415229316,-3.81672433495168));
#87796=CARTESIAN_POINT('Ctrl Pts',(17.5634294937014,-17.1880636691209,-3.81646850327567));
#87797=CARTESIAN_POINT('Ctrl Pts',(17.5533063828614,-17.1948105007833,-3.81572654851427));
#87798=CARTESIAN_POINT('Ctrl Pts',(17.5467081660945,-17.199262013236,-3.81523867130936));
#87799=CARTESIAN_POINT('Ctrl Pts',(17.5025881638244,-17.2293911872176,-3.81194846959107));
#87800=CARTESIAN_POINT('Ctrl Pts',(17.4658797455245,-17.2562327482212,-3.80907482768865));
#87801=CARTESIAN_POINT('Ctrl Pts',(17.3337634640967,-17.3595270044605,-3.79830199559183));
#87802=CARTESIAN_POINT('Ctrl Pts',(17.2441660399604,-17.4430183007227,-3.79014604798256));
#87803=CARTESIAN_POINT('Ctrl Pts',(17.0664194241312,-17.6400024163357,-3.77268281766358));
#87804=CARTESIAN_POINT('Ctrl Pts',(16.9815645504966,-17.755694625775,-3.76347483767858));
#87805=CARTESIAN_POINT('Ctrl Pts',(16.901795132617,-17.8913786301542,-3.75386464117407));
#87806=CARTESIAN_POINT('Ctrl Pts',(16.8946919720711,-17.9037450881326,-3.75299843143494));
#87807=CARTESIAN_POINT('Ctrl Pts',(16.8835815735337,-17.9235487443865,-3.75162638229171));
#87808=CARTESIAN_POINT('Ctrl Pts',(16.8794930478376,-17.9309396169716,-3.75111762977918));
#87809=CARTESIAN_POINT('Ctrl Pts',(16.8723579144689,-17.9440221148231,-3.75022284251099));
#87810=CARTESIAN_POINT('Ctrl Pts',(16.8692929236678,-17.9497035405955,-3.74983615435323));
#87811=CARTESIAN_POINT('Ctrl Pts',(16.8630050086398,-17.9614878232486,-3.74903797206499));
#87812=CARTESIAN_POINT('Ctrl Pts',(16.8597858409595,-17.9675926057907,-3.74862661474516));
#87813=CARTESIAN_POINT('Ctrl Pts',(16.8515946320148,-17.98331212891,-3.74757279810752));
#87814=CARTESIAN_POINT('Ctrl Pts',(16.8466663336164,-17.9929495324342,-3.74693188645952));
#87815=CARTESIAN_POINT('Ctrl Pts',(16.8263674565624,-18.0334069568143,-3.74426243128477));
#87816=CARTESIAN_POINT('Ctrl Pts',(16.8116756834781,-18.0645629483003,-3.74225761538301));
#87817=CARTESIAN_POINT('Ctrl Pts',(16.7753496865696,-18.1467376515201,-3.73708924114751));
#87818=CARTESIAN_POINT('Ctrl Pts',(16.7549461831935,-18.1982724997234,-3.73396556158161));
#87819=CARTESIAN_POINT('Ctrl Pts',(16.7029519421197,-18.3463289493196,-3.72524230346317));
#87820=CARTESIAN_POINT('Ctrl Pts',(16.6762484995271,-18.4444043621154,-3.71976223416452));
#87821=CARTESIAN_POINT('Ctrl Pts',(16.6333350831171,-18.6629057711412,-3.70765435626206));
#87822=CARTESIAN_POINT('Ctrl Pts',(16.6202380799738,-18.7835631244798,-3.7010311353847));
#87823=CARTESIAN_POINT('Ctrl Pts',(16.6172719941243,-18.9161664058184,-3.69321455419334));
#87824=CARTESIAN_POINT('Ctrl Pts',(16.6171084528581,-18.9276758995571,-3.69253161992972));
#87825=CARTESIAN_POINT('Ctrl Pts',(16.6170172171078,-18.9427485195498,-3.69163072932575));
#87826=CARTESIAN_POINT('Ctrl Pts',(16.6170046457328,-18.9463111909341,-3.69141731051467));
#87827=CARTESIAN_POINT('Ctrl Pts',(16.6170002823543,-18.9506557850236,-3.69115645016002));
#87828=CARTESIAN_POINT('Ctrl Pts',(16.6169999302637,-18.9514377208871,-3.69110947701853));
#87829=CARTESIAN_POINT('Ctrl Pts',(16.6170000113955,-18.952219655168,-3.69106248006748));
#87830=CARTESIAN_POINT('Ctrl Pts',(16.6170000023184,-18.952099076172,-3.6890562790225));
#87831=CARTESIAN_POINT('Ctrl Pts',(16.6170002492315,-18.9573749670544,-3.68873698393553));
#87832=CARTESIAN_POINT('Ctrl Pts',(16.6170202186042,-18.9626508039048,-3.68841768884856));
#87833=CARTESIAN_POINT('Ctrl Pts',(16.6170599094811,-18.9679264921966,-3.68809839376159));
#87834=CARTESIAN_POINT('Ctrl Pts',(16.6176052825337,-19.0404171615204,-3.6837111151193));
#87835=CARTESIAN_POINT('Ctrl Pts',(16.6218794874508,-19.1130212561194,-3.67932383647701));
#87836=CARTESIAN_POINT('Ctrl Pts',(16.6298970753153,-19.1853235571758,-3.67493655783472));
#87837=CARTESIAN_POINT('Ctrl Pts',(16.6379042320844,-19.2575317910134,-3.67055498715875));
#87838=CARTESIAN_POINT('Ctrl Pts',(16.6496450608728,-19.3294385348527,-3.66617341648278));
#87839=CARTESIAN_POINT('Ctrl Pts',(16.6650821233697,-19.4006288218111,-3.66179184580682));
#87840=CARTESIAN_POINT('Ctrl Pts',(16.6805014135,-19.4717371488836,-3.65741531954138));
#87841=CARTESIAN_POINT('Ctrl Pts',(16.699608383448,-19.5421301883611,-3.65303879327594));
#87842=CARTESIAN_POINT('Ctrl Pts',(16.7223140614304,-19.6114002461034,-3.64866226701051));
#87843=CARTESIAN_POINT('Ctrl Pts',(16.729642720702,-19.633758382747,-3.64724966573001));
#87844=CARTESIAN_POINT('Ctrl Pts',(16.7373458912453,-19.6559996038205,-3.64583706444951));
#87845=CARTESIAN_POINT('Ctrl Pts',(16.7454194499637,-19.6781104571739,-3.64442446316901));
#87846=CARTESIAN_POINT('Origin',(18.734,-18.952,0.));
#87847=CARTESIAN_POINT('',(16.7477770216415,-19.6772709618372,-2.84456321880205));
#87848=CARTESIAN_POINT('',(16.7454194663415,-19.6781105020273,-3.06515442754877));
#87849=CARTESIAN_POINT('',(16.7454194499637,-19.6781104571739,0.));
#87850=CARTESIAN_POINT('Ctrl Pts',(16.7454194663415,-19.6781105020273,-3.06515442754877));
#87851=CARTESIAN_POINT('Ctrl Pts',(16.6929878119308,-19.5345172513892,-3.0751266878066));
#87852=CARTESIAN_POINT('Ctrl Pts',(16.6562469386904,-19.3856243212607,-3.08537383313559));
#87853=CARTESIAN_POINT('Ctrl Pts',(16.6280919228878,-19.1761614896224,-3.09899375775158));
#87854=CARTESIAN_POINT('Ctrl Pts',(16.6227108922585,-19.118001419432,-3.10269879205228));
#87855=CARTESIAN_POINT('Ctrl Pts',(16.6179213238052,-19.0239677147122,-3.10855848048557));
#87856=CARTESIAN_POINT('Ctrl Pts',(16.6170073709165,-18.988204547134,-3.11075698713295));
#87857=CARTESIAN_POINT('Ctrl Pts',(16.6169977968599,-18.9414601925486,-3.11359307297547));
#87858=CARTESIAN_POINT('Ctrl Pts',(16.6170808697555,-18.9304867773714,-3.11425616960496));
#87859=CARTESIAN_POINT('Ctrl Pts',(16.6173556709538,-18.9125808571879,-3.11533391888877));
#87860=CARTESIAN_POINT('Ctrl Pts',(16.6174961453154,-18.9056478761124,-3.11575016938094));
#87861=CARTESIAN_POINT('Ctrl Pts',(16.6178328490637,-18.8922747946274,-3.11655110933349));
#87862=CARTESIAN_POINT('Ctrl Pts',(16.618024418735,-18.8858346634128,-3.11693594024069));
#87863=CARTESIAN_POINT('Ctrl Pts',(16.61853734898,-18.8708874658032,-3.11782711206487));
#87864=CARTESIAN_POINT('Ctrl Pts',(16.6188806299516,-18.8623812255126,-3.11833276088101));
#87865=CARTESIAN_POINT('Ctrl Pts',(16.6201365679445,-18.8353134801192,-3.11993715889321));
#87866=CARTESIAN_POINT('Ctrl Pts',(16.6212423392476,-18.8167614964382,-3.12102985744796));
#87867=CARTESIAN_POINT('Ctrl Pts',(16.6243860783612,-18.7735960961615,-3.12355754005255));
#87868=CARTESIAN_POINT('Ctrl Pts',(16.6266107576611,-18.7489987587108,-3.12498672114695));
#87869=CARTESIAN_POINT('Ctrl Pts',(16.6359173801211,-18.66291851234,-3.12995531942993));
#87870=CARTESIAN_POINT('Ctrl Pts',(16.6452643311255,-18.6017101858117,-3.13342815559401));
#87871=CARTESIAN_POINT('Ctrl Pts',(16.6848813788517,-18.4015335039668,-3.14471623957749));
#87872=CARTESIAN_POINT('Ctrl Pts',(16.7264586032257,-18.2652135679846,-3.15226968718797));
#87873=CARTESIAN_POINT('Ctrl Pts',(16.8104679516061,-18.0646549989625,-3.16430895658454));
#87874=CARTESIAN_POINT('Ctrl Pts',(16.8432342673644,-17.9968251012381,-3.16856362054279));
#87875=CARTESIAN_POINT('Ctrl Pts',(16.884114370491,-17.9225816389908,-3.17358677619475));
#87876=CARTESIAN_POINT('Ctrl Pts',(16.888746046659,-17.9143021420719,-3.17415227598234));
#87877=CARTESIAN_POINT('Ctrl Pts',(16.895695423448,-17.9020732166805,-3.17499587372488));
#87878=CARTESIAN_POINT('Ctrl Pts',(16.8979706149233,-17.8980995954386,-3.17527130581961));
#87879=CARTESIAN_POINT('Ctrl Pts',(16.9020434262671,-17.8910396478425,-3.17576307170795));
#87880=CARTESIAN_POINT('Ctrl Pts',(16.9038359826543,-17.887950458731,-3.17597907716988));
#87881=CARTESIAN_POINT('Ctrl Pts',(16.9077088544987,-17.881314912925,-3.17644484920485));
#87882=CARTESIAN_POINT('Ctrl Pts',(16.9097916553653,-17.8777701277092,-3.17669477185982));
#87883=CARTESIAN_POINT('Ctrl Pts',(16.9155744490497,-17.8679935233195,-3.17738706504045));
#87884=CARTESIAN_POINT('Ctrl Pts',(16.9192960972128,-17.8617746712057,-3.17783080994103));
#87885=CARTESIAN_POINT('Ctrl Pts',(16.9399457462415,-17.8276679181774,-3.18028261422351));
#87886=CARTESIAN_POINT('Ctrl Pts',(16.9574837344677,-17.800156702163,-3.18232721188365));
#87887=CARTESIAN_POINT('Ctrl Pts',(17.0662163423063,-17.6379850569763,-3.19473510295501));
#87888=CARTESIAN_POINT('Ctrl Pts',(17.1720438904539,-17.5137960322802,-3.20568689909559));
#87889=CARTESIAN_POINT('Ctrl Pts',(17.3764983370213,-17.3233449860685,-3.22393799246217));
#87890=CARTESIAN_POINT('Ctrl Pts',(17.468403675699,-17.2509410167191,-3.23137711130904));
#87891=CARTESIAN_POINT('Ctrl Pts',(17.5777443369557,-17.1785947960711,-3.23938256626324));
#87892=CARTESIAN_POINT('Ctrl Pts',(17.589740723416,-17.170830749392,-3.24025052130294));
#87893=CARTESIAN_POINT('Ctrl Pts',(17.6089588009776,-17.1586671313934,-3.24162480304224));
#87894=CARTESIAN_POINT('Ctrl Pts',(17.6161296676214,-17.1541884413684,-3.24213405763158));
#87895=CARTESIAN_POINT('Ctrl Pts',(17.6288239824135,-17.1463653029585,-3.24302942879101));
#87896=CARTESIAN_POINT('Ctrl Pts',(17.6343362260577,-17.1430029644247,-3.24341620145572));
#87897=CARTESIAN_POINT('Ctrl Pts',(17.6457691797278,-17.1361007005969,-3.24421427160267));
#87898=CARTESIAN_POINT('Ctrl Pts',(17.6516919883643,-17.1325643860132,-3.24462543368715));
#87899=CARTESIAN_POINT('Ctrl Pts',(17.6669394887133,-17.1235614048688,-3.24567815661206));
#87900=CARTESIAN_POINT('Ctrl Pts',(17.6762890268787,-17.1181370457937,-3.24631817607566));
#87901=CARTESIAN_POINT('Ctrl Pts',(17.7154849584691,-17.0957960615331,-3.24897894475541));
#87902=CARTESIAN_POINT('Ctrl Pts',(17.7456997747558,-17.0795340290371,-3.25097616290278));
#87903=CARTESIAN_POINT('Ctrl Pts',(17.82544479408,-17.0390824939131,-3.25612052479162));
#87904=CARTESIAN_POINT('Ctrl Pts',(17.8755487072211,-17.0160795546499,-3.25922827383286));
#87905=CARTESIAN_POINT('Ctrl Pts',(18.0275780153212,-16.9533468909902,-3.26837301596235));
#87906=CARTESIAN_POINT('Ctrl Pts',(18.1317424557326,-16.9195303189857,-3.27426128077102));
#87907=CARTESIAN_POINT('Ctrl Pts',(18.2827866595482,-16.8831324711306,-3.28272016959122));
#87908=CARTESIAN_POINT('Ctrl Pts',(18.3278589516331,-16.8738143642051,-3.28523621522726));
#87909=CARTESIAN_POINT('Ctrl Pts',(18.3949986035987,-16.8622017907978,-3.28901509345587));
#87910=CARTESIAN_POINT('Ctrl Pts',(18.4168568565131,-16.85877314151,-3.2902502108794));
#87911=CARTESIAN_POINT('Ctrl Pts',(18.4897456676548,-16.8485077904856,-3.29439632997475));
#87912=CARTESIAN_POINT('Ctrl Pts',(18.5409676587761,-16.8431905624212,-3.29735450970791));
#87913=CARTESIAN_POINT('Ctrl Pts',(18.6009479067983,-16.8391675926959,-3.30092249109881));
#87914=CARTESIAN_POINT('Ctrl Pts',(18.6095713250742,-16.8386422120369,-3.30143796809104));
#87915=CARTESIAN_POINT('Ctrl Pts',(18.6226566738216,-16.8379253543991,-3.3022242864335));
#87916=CARTESIAN_POINT('Ctrl Pts',(18.6271165120674,-16.8376951821878,-3.30249301091803));
#87917=CARTESIAN_POINT('Ctrl Pts',(18.6351357098835,-16.8373067488918,-3.30297756050041));
#87918=CARTESIAN_POINT('Ctrl Pts',(18.6386947665896,-16.8371433603391,-3.30319309540201));
#87919=CARTESIAN_POINT('Ctrl Pts',(18.6464437549328,-16.8368072218244,-3.3036634342197));
#87920=CARTESIAN_POINT('Ctrl Pts',(18.650633738967,-16.8366379386228,-3.30391842431085));
#87921=CARTESIAN_POINT('Ctrl Pts',(18.6624420185504,-16.8361959995301,-3.30463888035573));
#87922=CARTESIAN_POINT('Ctrl Pts',(18.6700612330957,-16.8359520461146,-3.30510590624734));
#87923=CARTESIAN_POINT('Ctrl Pts',(18.7164060655347,-16.8347186983736,-3.30795908111973));
#87924=CARTESIAN_POINT('Ctrl Pts',(18.7551489221768,-16.8347513273524,-3.3103969363245));
#87925=CARTESIAN_POINT('Ctrl Pts',(18.8845066755227,-16.8384108649624,-3.31866554155012));
#87926=CARTESIAN_POINT('Ctrl Pts',(18.9748834288029,-16.8467958622333,-3.32465014995911));
#87927=CARTESIAN_POINT('Ctrl Pts',(19.1307356709466,-16.8714243693294,-3.33507705698038));
#87928=CARTESIAN_POINT('Ctrl Pts',(19.1964996704821,-16.8850484410584,-3.33951160002356));
#87929=CARTESIAN_POINT('Ctrl Pts',(19.3726439820372,-16.9303689816104,-3.35138287256244));
#87930=CARTESIAN_POINT('Ctrl Pts',(19.4812855501041,-16.9679561905951,-3.35868685817627));
#87931=CARTESIAN_POINT('Ctrl Pts',(19.5994118911057,-17.0199144461165,-3.36656624067994));
#87932=CARTESIAN_POINT('Ctrl Pts',(19.6124062894499,-17.0257874636828,-3.36743236959852));
#87933=CARTESIAN_POINT('Ctrl Pts',(19.6330013210753,-17.0353474606847,-3.36880431539321));
#87934=CARTESIAN_POINT('Ctrl Pts',(19.6406407670703,-17.038949333009,-3.36931304469359));
#87935=CARTESIAN_POINT('Ctrl Pts',(19.6540808180703,-17.0453846850884,-3.37020780503022));
#87936=CARTESIAN_POINT('Ctrl Pts',(19.6598903629394,-17.0481991416946,-3.37059448934382));
#87937=CARTESIAN_POINT('Ctrl Pts',(19.6718842896612,-17.054077532836,-3.37139267702283));
#87938=CARTESIAN_POINT('Ctrl Pts',(19.6780667506292,-17.0571452287181,-3.37180404351184));
#87939=CARTESIAN_POINT('Ctrl Pts',(19.6939072324825,-17.0651019419504,-3.37285791127719));
#87940=CARTESIAN_POINT('Ctrl Pts',(19.703543032472,-17.070034938896,-3.37349886458995));
#87941=CARTESIAN_POINT('Ctrl Pts',(19.7436809711016,-17.09097343798,-3.37616872547413));
#87942=CARTESIAN_POINT('Ctrl Pts',(19.7738290176351,-17.1076488021566,-3.37817389622223));
#87943=CARTESIAN_POINT('Ctrl Pts',(19.8513821287972,-17.1530510833581,-3.3833433927107));
#87944=CARTESIAN_POINT('Ctrl Pts',(19.8980906208808,-17.1829172694466,-3.38646781697899));
#87945=CARTESIAN_POINT('Ctrl Pts',(20.0335283536706,-17.2772079866678,-3.39564163839637));
#87946=CARTESIAN_POINT('Ctrl Pts',(20.1184839030284,-17.3467251308334,-3.40154240748138));
#87947=CARTESIAN_POINT('Ctrl Pts',(20.2426880705409,-17.4655844554062,-3.41090353833762));
#87948=CARTESIAN_POINT('Ctrl Pts',(20.2857763120577,-17.5106255145485,-3.41431590378571));
#87949=CARTESIAN_POINT('Ctrl Pts',(20.3638835055738,-17.5998403304361,-3.42096846609233));
#87950=CARTESIAN_POINT('Ctrl Pts',(20.3992470852891,-17.6436395828636,-3.42419095948977));
#87951=CARTESIAN_POINT('Ctrl Pts',(20.4380913535933,-17.6958791140761,-3.42805324093422));
#87952=CARTESIAN_POINT('Ctrl Pts',(20.4433174521482,-17.7030000548105,-3.42858011390047));
#87953=CARTESIAN_POINT('Ctrl Pts',(20.4511428251084,-17.7138037977882,-3.42938041123623));
#87954=CARTESIAN_POINT('Ctrl Pts',(20.4537752252823,-17.7174626410534,-3.42965160424009));
#87955=CARTESIAN_POINT('Ctrl Pts',(20.4584690464068,-17.7240308546511,-3.43013878125471));
#87956=CARTESIAN_POINT('Ctrl Pts',(20.4605348191367,-17.7269370497912,-3.4303544610024));
#87957=CARTESIAN_POINT('Ctrl Pts',(20.4649957846162,-17.7332465742658,-3.43082299075424));
#87958=CARTESIAN_POINT('Ctrl Pts',(20.4673882545621,-17.7366517053306,-3.43107601535337));
#87959=CARTESIAN_POINT('Ctrl Pts',(20.4740509429589,-17.7461942037436,-3.43178550586733));
#87960=CARTESIAN_POINT('Ctrl Pts',(20.4782986614297,-17.7523471009167,-3.43224345821451));
#87961=CARTESIAN_POINT('Ctrl Pts',(20.5029243404329,-17.788425139012,-3.43493088254932));
#87962=CARTESIAN_POINT('Ctrl Pts',(20.5225632323499,-17.8188446795622,-3.43720546748143));
#87963=CARTESIAN_POINT('Ctrl Pts',(20.5834759133727,-17.9187261157347,-3.44466425493239));
#87964=CARTESIAN_POINT('Ctrl Pts',(20.6215550303776,-17.990048678822,-3.4499732776991));
#87965=CARTESIAN_POINT('Ctrl Pts',(20.7329367226437,-18.2308858046551,-3.46749356162998));
#87966=CARTESIAN_POINT('Ctrl Pts',(20.7881878558816,-18.4078555835435,-3.47965047893929));
#87967=CARTESIAN_POINT('Ctrl Pts',(20.823580026576,-18.6116510388398,-3.4923723548316));
#87968=CARTESIAN_POINT('Ctrl Pts',(20.8270351885077,-18.6335885343617,-3.49372726039878));
#87969=CARTESIAN_POINT('Ctrl Pts',(20.8313312375178,-18.6639678923453,-3.49558414298879));
#87970=CARTESIAN_POINT('Ctrl Pts',(20.8324674404825,-18.6723659187258,-3.49609541872434));
#87971=CARTESIAN_POINT('Ctrl Pts',(20.8343324294193,-18.6868025691583,-3.49697089150009));
#87972=CARTESIAN_POINT('Ctrl Pts',(20.8350856687601,-18.6928378786808,-3.49733585726129));
#87973=CARTESIAN_POINT('Ctrl Pts',(20.8365837295177,-18.7052770325794,-3.498085985456));
#87974=CARTESIAN_POINT('Ctrl Pts',(20.8373253294104,-18.7116812067996,-3.49847104254219));
#87975=CARTESIAN_POINT('Ctrl Pts',(20.8389811831568,-18.7265756518922,-3.49936398498728));
#87976=CARTESIAN_POINT('Ctrl Pts',(20.8398733486626,-18.7350683038006,-3.49987116946171));
#87977=CARTESIAN_POINT('Ctrl Pts',(20.8425577771957,-18.7622007744136,-3.50148543461715));
#87978=CARTESIAN_POINT('Ctrl Pts',(20.8441541585666,-18.7808593962848,-3.50258635738023));
#87979=CARTESIAN_POINT('Ctrl Pts',(20.8472984892433,-18.8244061696206,-3.50513586265569));
#87980=CARTESIAN_POINT('Ctrl Pts',(20.8486547298727,-18.8493056134864,-3.50657850053666));
#87981=CARTESIAN_POINT('Ctrl Pts',(20.8518764099744,-18.9369379110832,-3.51160921368987));
#87982=CARTESIAN_POINT('Ctrl Pts',(20.8513923696498,-18.9997262945109,-3.51512876620645));
#87983=CARTESIAN_POINT('Ctrl Pts',(20.8429272825505,-19.1618232678387,-3.52410228098342));
#87984=CARTESIAN_POINT('Ctrl Pts',(20.8307287512515,-19.2607541322247,-3.52946528721185));
#87985=CARTESIAN_POINT('Ctrl Pts',(20.7977315712765,-19.4294192163148,-3.5388261351708));
#87986=CARTESIAN_POINT('Ctrl Pts',(20.7802235413917,-19.4996175919569,-3.54279176801564));
#87987=CARTESIAN_POINT('Ctrl Pts',(20.745811363295,-19.6126083085533,-3.54947847157277));
#87988=CARTESIAN_POINT('Ctrl Pts',(20.7310441134659,-19.6559903652426,-3.55212194170258));
#87989=CARTESIAN_POINT('Ctrl Pts',(20.7121911226638,-19.7059940873989,-3.55529550344302));
#87990=CARTESIAN_POINT('Ctrl Pts',(20.7094611695431,-19.7131178392859,-3.55575067104188));
#87991=CARTESIAN_POINT('Ctrl Pts',(20.705020057454,-19.7245219619774,-3.55648446637239));
#87992=CARTESIAN_POINT('Ctrl Pts',(20.7033332897576,-19.7288118443712,-3.55676166916453));
#87993=CARTESIAN_POINT('Ctrl Pts',(20.7003103909126,-19.7364267253825,-3.55725586860305));
#87994=CARTESIAN_POINT('Ctrl Pts',(20.6989798136129,-19.7397538783283,-3.55747252923452));
#87995=CARTESIAN_POINT('Ctrl Pts',(20.6961295307234,-19.7468289504677,-3.55793482807171));
#87996=CARTESIAN_POINT('Ctrl Pts',(20.6946075546993,-19.7505758396426,-3.55818059702074));
#87997=CARTESIAN_POINT('Ctrl Pts',(20.6904434649384,-19.7607435791892,-3.55885003843898));
#87998=CARTESIAN_POINT('Ctrl Pts',(20.6877805113774,-19.7671557634323,-3.55927494237368));
#87999=CARTESIAN_POINT('Ctrl Pts',(20.6740339861199,-19.7998019850031,-3.56145175709801));
#88000=CARTESIAN_POINT('Ctrl Pts',(20.6624539592293,-19.8258221875199,-3.56323137952491));
#88001=CARTESIAN_POINT('Ctrl Pts',(20.6268633544729,-19.9016383523107,-3.56853243317356));
#88002=CARTESIAN_POINT('Ctrl Pts',(20.6014240454178,-19.9507348377574,-3.57211444958112));
#88003=CARTESIAN_POINT('Ctrl Pts',(20.5047213131587,-20.1207255460475,-3.58492306465189));
#88004=CARTESIAN_POINT('Ctrl Pts',(20.4233892784576,-20.2354883471711,-3.59429839358696));
#88005=CARTESIAN_POINT('Ctrl Pts',(20.2725645290536,-20.4088863033187,-3.6091303704621));
#88006=CARTESIAN_POINT('Ctrl Pts',(20.2096010753973,-20.4726260587315,-3.61476942843988));
#88007=CARTESIAN_POINT('Ctrl Pts',(20.1325547703226,-20.5413147378914,-3.62106716907435));
#88008=CARTESIAN_POINT('Ctrl Pts',(20.1222376773322,-20.55033442895,-3.62189908283746));
#88009=CARTESIAN_POINT('Ctrl Pts',(20.1055446783812,-20.5646446632317,-3.62322717749021));
#88010=CARTESIAN_POINT('Ctrl Pts',(20.099224162141,-20.5699989508024,-3.62372598789833));
#88011=CARTESIAN_POINT('Ctrl Pts',(20.0879418613428,-20.5794433261227,-3.6246092828644));
#88012=CARTESIAN_POINT('Ctrl Pts',(20.0829925918295,-20.5835481397254,-3.62499436775926));
#88013=CARTESIAN_POINT('Ctrl Pts',(20.0726375354417,-20.5920570616006,-3.62579512269359));
#88014=CARTESIAN_POINT('Ctrl Pts',(20.0672285306139,-20.596457145548,-3.62621062672019));
#88015=CARTESIAN_POINT('Ctrl Pts',(20.0531161477256,-20.6078218017888,-3.62728758829109));
#88016=CARTESIAN_POINT('Ctrl Pts',(20.0443792552369,-20.6147445579825,-3.6279473628926));
#88017=CARTESIAN_POINT('Ctrl Pts',(20.006115289842,-20.6445744417216,-3.63080729705498));
#88018=CARTESIAN_POINT('Ctrl Pts',(19.976038190382,-20.6667673127824,-3.63297919132641));
#88019=CARTESIAN_POINT('Ctrl Pts',(19.8944835086819,-20.7236714762194,-3.63868555838165));
#88020=CARTESIAN_POINT('Ctrl Pts',(19.842039305766,-20.7569353336805,-3.64216835312113));
#88021=CARTESIAN_POINT('Ctrl Pts',(19.7066140021285,-20.8347010921331,-3.65080589663979));
#88022=CARTESIAN_POINT('Ctrl Pts',(19.6219877195809,-20.8760633537659,-3.65588386369722));
#88023=CARTESIAN_POINT('Ctrl Pts',(19.4209112203347,-20.9582410457526,-3.66770034735924));
#88024=CARTESIAN_POINT('Ctrl Pts',(19.3031012787516,-20.9947836263324,-3.67444428234046));
#88025=CARTESIAN_POINT('Ctrl Pts',(19.1735781040909,-21.0228812693016,-3.68230000478838));
#88026=CARTESIAN_POINT('Ctrl Pts',(19.1643381602837,-21.0248210731927,-3.68286282137508));
#88027=CARTESIAN_POINT('Ctrl Pts',(19.1506071096526,-21.0276079592811,-3.68370317429446));
#88028=CARTESIAN_POINT('Ctrl Pts',(19.146125590979,-21.0285024393932,-3.68397807446866));
#88029=CARTESIAN_POINT('Ctrl Pts',(19.1381372401925,-21.030069980058,-3.68446925961072));
#88030=CARTESIAN_POINT('Ctrl Pts',(19.1346315676104,-21.0307486855619,-3.68468521926273));
#88031=CARTESIAN_POINT('Ctrl Pts',(19.1270798011099,-21.0321909102926,-3.6851513149039));
#88032=CARTESIAN_POINT('Ctrl Pts',(19.1230332507196,-21.0329514848914,-3.68540160920954));
#88033=CARTESIAN_POINT('Ctrl Pts',(19.1118310092363,-21.0350232000108,-3.68609595633987));
#88034=CARTESIAN_POINT('Ctrl Pts',(19.1046708183316,-21.0363092534995,-3.68654139671802));
#88035=CARTESIAN_POINT('Ctrl Pts',(19.0661909303955,-21.0430161400399,-3.68894348415039));
#88036=CARTESIAN_POINT('Ctrl Pts',(19.034760551346,-21.0477676758665,-3.69093469815174));
#88037=CARTESIAN_POINT('Ctrl Pts',(18.8413360407889,-21.0725685285995,-3.70331903437222));
#88038=CARTESIAN_POINT('Ctrl Pts',(18.677582087001,-21.0745335751913,-3.71431231851128));
#88039=CARTESIAN_POINT('Ctrl Pts',(18.3988799792387,-21.0455775596452,-3.73261605511738));
#88040=CARTESIAN_POINT('Ctrl Pts',(18.2837177635398,-21.0238653845563,-3.7400678636223));
#88041=CARTESIAN_POINT('Ctrl Pts',(18.157146194391,-20.9889420546946,-3.74808512920842));
#88042=CARTESIAN_POINT('Ctrl Pts',(18.1434080704915,-20.9850013368793,-3.7489532384406));
#88043=CARTESIAN_POINT('Ctrl Pts',(18.1216072735578,-20.9785082378315,-3.75032771740004));
#88044=CARTESIAN_POINT('Ctrl Pts',(18.1135183529135,-20.9760461996375,-3.75083701632456));
#88045=CARTESIAN_POINT('Ctrl Pts',(18.0992786498256,-20.9716186516714,-3.75173243905438));
#88046=CARTESIAN_POINT('Ctrl Pts',(18.0931217435938,-20.9696733512748,-3.75211921919221));
#88047=CARTESIAN_POINT('Ctrl Pts',(18.0804060419492,-20.9655916958743,-3.75291727950037));
#88048=CARTESIAN_POINT('Ctrl Pts',(18.0738485877795,-20.963451390009,-3.7533284243975));
#88049=CARTESIAN_POINT('Ctrl Pts',(18.0570440857223,-20.9578754926461,-3.75438105103633));
#88050=CARTESIAN_POINT('Ctrl Pts',(18.0468125934279,-20.9543933870944,-3.75502099195474));
#88051=CARTESIAN_POINT('Ctrl Pts',(18.0048406986407,-20.9397494122098,-3.75764268417117));
#88052=CARTESIAN_POINT('Ctrl Pts',(17.9733408712749,-20.9279096356135,-3.75960190936131));
#88053=CARTESIAN_POINT('Ctrl Pts',(17.8921213235861,-20.8951514618229,-3.76464267812894));
#88054=CARTESIAN_POINT('Ctrl Pts',(17.8428941577103,-20.8730747767913,-3.76768656685087));
#88055=CARTESIAN_POINT('Ctrl Pts',(17.6804863961486,-20.7926526121985,-3.7777732338643));
#88056=CARTESIAN_POINT('Ctrl Pts',(17.5717408942585,-20.7259918550786,-3.78458690825506));
#88057=CARTESIAN_POINT('Ctrl Pts',(17.3877478764065,-20.5889848486864,-3.79713119948763));
#88058=CARTESIAN_POINT('Ctrl Pts',(17.3103837739456,-20.5221673271203,-3.80279980197864));
#88059=CARTESIAN_POINT('Ctrl Pts',(17.2312943914325,-20.4431937398383,-3.80942141152686));
#88060=CARTESIAN_POINT('Ctrl Pts',(17.2244840385472,-20.4362993194805,-3.80999891040315));
#88061=CARTESIAN_POINT('Ctrl Pts',(17.2144981906804,-20.4260504008823,-3.81085700423173));
#88062=CARTESIAN_POINT('Ctrl Pts',(17.2112858427278,-20.4227317658848,-3.81113479857101));
#88063=CARTESIAN_POINT('Ctrl Pts',(17.2056059510784,-20.4168253876997,-3.81162915932021));
#88064=CARTESIAN_POINT('Ctrl Pts',(17.2031340761522,-20.4142418774679,-3.81184538401416));
#88065=CARTESIAN_POINT('Ctrl Pts',(17.1978517143835,-20.4086928766961,-3.81230979083259));
#88066=CARTESIAN_POINT('Ctrl Pts',(17.1950433058898,-20.4057255536794,-3.81255811939621));
#88067=CARTESIAN_POINT('Ctrl Pts',(17.1892976396484,-20.3996194587759,-3.81306906338758));
#88068=CARTESIAN_POINT('Ctrl Pts',(17.1863613190114,-20.3964798343598,-3.81333174696066));
#88069=CARTESIAN_POINT('Ctrl Pts',(17.1729076005358,-20.3820064999248,-3.81454244666627));
#88070=CARTESIAN_POINT('Ctrl Pts',(17.1625053224303,-20.3705670643121,-3.81549867412406));
#88071=CARTESIAN_POINT('Ctrl Pts',(17.0941973460345,-20.2937750436813,-3.82190711715058));
#88072=CARTESIAN_POINT('Ctrl Pts',(17.0402625680135,-20.2250135063294,-3.82759172307141));
#88073=CARTESIAN_POINT('Ctrl Pts',(16.9494514018129,-20.0932138424625,-3.83812736757958));
#88074=CARTESIAN_POINT('Ctrl Pts',(16.9112865270765,-20.0312119709267,-3.84295320930795));
#88075=CARTESIAN_POINT('Ctrl Pts',(16.8741060748315,-19.9631905116076,-3.84805125670443));
#88076=CARTESIAN_POINT('Ctrl Pts',(16.8718368428655,-19.9590054816583,-3.84836415855552));
#88077=CARTESIAN_POINT('Ctrl Pts',(16.8216174704287,-19.8656381923011,-3.8553278644878));
#88078=CARTESIAN_POINT('Ctrl Pts',(16.7801280770989,-19.773166078775,-3.86186882433325));
#88079=CARTESIAN_POINT('Ctrl Pts',(16.7454195176904,-19.6781106426554,-3.8681936027756));
#88080=CARTESIAN_POINT('',(16.6170008393112,-18.9501148891278,-2.8890562790225));
#88081=CARTESIAN_POINT('Ctrl Pts',(16.7454194499637,-19.6781104571739,-3.64442446316901));
#88082=CARTESIAN_POINT('Ctrl Pts',(16.7704138786351,-19.7465620738999,-3.64005127865668));
#88083=CARTESIAN_POINT('Ctrl Pts',(16.7989618298144,-19.8137628460192,-3.63567809414436));
#88084=CARTESIAN_POINT('Ctrl Pts',(16.8309082925844,-19.8793246212443,-3.63130490963203));
#88085=CARTESIAN_POINT('Ctrl Pts',(16.8628484343729,-19.9448734243051,-3.62693259040543));
#88086=CARTESIAN_POINT('Ctrl Pts',(16.8981855408596,-20.0087834410941,-3.62256027117883));
#88087=CARTESIAN_POINT('Ctrl Pts',(16.9367174467763,-20.0706887073167,-3.61818795195223));
#88088=CARTESIAN_POINT('Ctrl Pts',(16.9752544392512,-20.1326021455912,-3.61381505554016));
#88089=CARTESIAN_POINT('Ctrl Pts',(17.0169868114736,-20.1925098997059,-3.6094421591281));
#88090=CARTESIAN_POINT('Ctrl Pts',(17.0616685465372,-20.2500741541835,-3.60506926271603));
#88091=CARTESIAN_POINT('Ctrl Pts',(17.1063995656089,-20.3077019021036,-3.60069154299392));
#88092=CARTESIAN_POINT('Ctrl Pts',(17.1540861421439,-20.3629806112168,-3.59631382327181));
#88093=CARTESIAN_POINT('Ctrl Pts',(17.2044419174547,-20.4156055042669,-3.5919361035497));
#88094=CARTESIAN_POINT('Ctrl Pts',(17.2548300001719,-20.4682641605506,-3.58755557515729));
#88095=CARTESIAN_POINT('Ctrl Pts',(17.3078903383435,-20.5182652822583,-3.58317504676489));
#88096=CARTESIAN_POINT('Ctrl Pts',(17.3633016190121,-20.5653427869976,-3.57879451837249));
#88097=CARTESIAN_POINT('Ctrl Pts',(17.4188056844067,-20.6124991217751,-3.574406654901));
#88098=CARTESIAN_POINT('Ctrl Pts',(17.4766681642482,-20.6567217793341,-3.57001879142951));
#88099=CARTESIAN_POINT('Ctrl Pts',(17.5365374607371,-20.6977870623481,-3.56563092795801));
#88100=CARTESIAN_POINT('Ctrl Pts',(17.557951455484,-20.7124752548995,-3.56406148099873));
#88101=CARTESIAN_POINT('Ctrl Pts',(17.5796219547575,-20.7267599352232,-3.56249203403944));
#88102=CARTESIAN_POINT('Ctrl Pts',(17.6015321394765,-20.7406323112595,-3.56092258708016));
#88103=CARTESIAN_POINT('Ctrl Pts',(17.6627935078072,-20.7794197860744,-3.55653437814988));
#88104=CARTESIAN_POINT('Ctrl Pts',(17.7261694924202,-20.8151319931224,-3.55214616921959));
#88105=CARTESIAN_POINT('Ctrl Pts',(17.7913186157341,-20.8475318007774,-3.54775796028931));
#88106=CARTESIAN_POINT('Ctrl Pts',(17.856371046947,-20.8798835217459,-3.54337626418866));
#88107=CARTESIAN_POINT('Ctrl Pts',(17.9231909643684,-20.908932389527,-3.53899456808801));
#88108=CARTESIAN_POINT('Ctrl Pts',(17.9914091442166,-20.9344852637301,-3.53461287198736));
#88109=CARTESIAN_POINT('Ctrl Pts',(18.0595471622743,-20.9600081112723,-3.53023632472835));
#88110=CARTESIAN_POINT('Ctrl Pts',(18.129079729305,-20.982042957579,-3.52585977746933));
#88111=CARTESIAN_POINT('Ctrl Pts',(18.1996158698655,-21.0004439463799,-3.52148323021032));
#88112=CARTESIAN_POINT('Ctrl Pts',(18.2701072774307,-21.018833265541,-3.51710945849398));
#88113=CARTESIAN_POINT('Ctrl Pts',(18.3416005301147,-21.033593178237,-3.51273568677764));
#88114=CARTESIAN_POINT('Ctrl Pts',(18.4136889989953,-21.0446275021215,-3.5083619150613));
#88115=CARTESIAN_POINT('Ctrl Pts',(18.4857555311126,-21.0556584682242,-3.50398947429839));
#88116=CARTESIAN_POINT('Ctrl Pts',(18.5584164432973,-21.0629660233357,-3.49961703353548));
#88117=CARTESIAN_POINT('Ctrl Pts',(18.631256065406,-21.0665053047709,-3.49524459277256));
#88118=CARTESIAN_POINT('Ctrl Pts',(18.7040975500317,-21.0700446767059,-3.49087204020586));
#88119=CARTESIAN_POINT('Ctrl Pts',(18.7771172717475,-21.0698155622466,-3.48649948763916));
#88120=CARTESIAN_POINT('Ctrl Pts',(18.8498972932268,-21.0658251624538,-3.48212693507246));
#88121=CARTESIAN_POINT('Ctrl Pts',(18.9227528485576,-21.0618306212735,-3.47774984450578));
#88122=CARTESIAN_POINT('Ctrl Pts',(18.9953677242811,-21.0540670274162,-3.47337275393909));
#88123=CARTESIAN_POINT('Ctrl Pts',(19.0673276840493,-21.0425936130789,-3.46899566337241));
#88124=CARTESIAN_POINT('Ctrl Pts',(19.1393269438223,-21.0311139326842,-3.46461618231411));
#88125=CARTESIAN_POINT('Ctrl Pts',(19.2106701033903,-21.0159204984676,-3.46023670125581));
#88126=CARTESIAN_POINT('Ctrl Pts',(19.2809543980021,-20.997123440408,-3.45585722019751));
#88127=CARTESIAN_POINT('Ctrl Pts',(19.3513632710544,-20.9782930646891,-3.45146997653843));
#88128=CARTESIAN_POINT('Ctrl Pts',(19.420709071857,-20.9558464584345,-3.44708273287935));
#88129=CARTESIAN_POINT('Ctrl Pts',(19.4886059995044,-20.9299430693303,-3.44269548922027));
#88130=CARTESIAN_POINT('Ctrl Pts',(19.5347693678672,-20.912331260748,-3.43971258627975));
#88131=CARTESIAN_POINT('Ctrl Pts',(19.5802633709749,-20.8931225055476,-3.43672968333924));
#88132=CARTESIAN_POINT('Ctrl Pts',(19.6249733426256,-20.872378999763,-3.43374678039872));
#88133=CARTESIAN_POINT('Ctrl Pts',(19.6907470875159,-20.841862808246,-3.4293585714646));
#88134=CARTESIAN_POINT('Ctrl Pts',(19.7550796205686,-20.8079039749602,-3.42497036253047));
#88135=CARTESIAN_POINT('Ctrl Pts',(19.8175867162743,-20.7706612736609,-3.42058215359634));
#88136=CARTESIAN_POINT('Ctrl Pts',(19.8800010410864,-20.7334738467051,-3.41620045749183));
#88137=CARTESIAN_POINT('Ctrl Pts',(19.9405948958128,-20.6930124717672,-3.41181876138733));
#88138=CARTESIAN_POINT('Ctrl Pts',(19.9990060261196,-20.6494830643871,-3.40743706528282));
#88139=CARTESIAN_POINT('Ctrl Pts',(20.0573485186997,-20.6060048075249,-3.40306051801995));
#88140=CARTESIAN_POINT('Ctrl Pts',(20.1135129971335,-20.5594659667509,-3.39868397075708));
#88141=CARTESIAN_POINT('Ctrl Pts',(20.1671651917874,-20.5101163413073,-3.3943074234942));
#88142=CARTESIAN_POINT('Ctrl Pts',(20.2207833609993,-20.460798012679,-3.389933651774));
#88143=CARTESIAN_POINT('Ctrl Pts',(20.271892053496,-20.4086727619653,-3.38555988005379));
#88144=CARTESIAN_POINT('Ctrl Pts',(20.3201902946221,-20.35403043806,-3.38118610833359));
#88145=CARTESIAN_POINT('Ctrl Pts',(20.3684738384311,-20.2994047419976,-3.37681366756681));
#88146=CARTESIAN_POINT('Ctrl Pts',(20.4139483094908,-20.2422638546087,-3.37244122680004));
#88147=CARTESIAN_POINT('Ctrl Pts',(20.4563509910175,-20.1829330053829,-3.36806878603326));
#88148=CARTESIAN_POINT('Ctrl Pts',(20.4987547567854,-20.123600639061,-3.36369623346271));
#88149=CARTESIAN_POINT('Ctrl Pts',(20.5380862982223,-20.0620785933403,-3.35932368089216));
#88150=CARTESIAN_POINT('Ctrl Pts',(20.5741254487321,-19.9987221851707,-3.3549511283216));
#88151=CARTESIAN_POINT('Ctrl Pts',(20.6102020020313,-19.9353000233316,-3.35057403775111));
#88152=CARTESIAN_POINT('Ctrl Pts',(20.6429791031822,-19.8700401182239,-3.34619694718061));
#88153=CARTESIAN_POINT('Ctrl Pts',(20.67228233881,-19.8033228383271,-3.34181985661012));
#88154=CARTESIAN_POINT('Ctrl Pts',(20.7016015780221,-19.7365691216478,-3.33744037554803));
#88155=CARTESIAN_POINT('Ctrl Pts',(20.7274430033812,-19.6683568969028,-3.33306089448594));
#88156=CARTESIAN_POINT('Ctrl Pts',(20.7496812078499,-19.5990844367782,-3.32868141342385));
#88157=CARTESIAN_POINT('Ctrl Pts',(20.7719588293865,-19.5296891916842,-3.32429416976104));
#88158=CARTESIAN_POINT('Ctrl Pts',(20.790620352471,-19.4592304251149,-3.31990692609824));
#88159=CARTESIAN_POINT('Ctrl Pts',(20.8055910206615,-19.3881188405866,-3.31551968243543));
#88160=CARTESIAN_POINT('Ctrl Pts',(20.8157696323556,-19.3397698159036,-3.31253677952939));
#88161=CARTESIAN_POINT('Ctrl Pts',(20.8242431499885,-19.2911192245624,-3.30955387662334));
#88162=CARTESIAN_POINT('Ctrl Pts',(20.8310018039417,-19.2422971482213,-3.30657097371729));
#88163=CARTESIAN_POINT('Ctrl Pts',(20.8409445967654,-19.1704740021267,-3.30218276479086));
#88164=CARTESIAN_POINT('Ctrl Pts',(20.8472125720511,-19.0979992504157,-3.29779455586442));
#88165=CARTESIAN_POINT('Ctrl Pts',(20.8497312594192,-19.0252819071575,-3.29340634693799));
#88166=CARTESIAN_POINT('Ctrl Pts',(20.8522462086376,-18.9526724884933,-3.28902465084117));
#88167=CARTESIAN_POINT('Ctrl Pts',(20.8510228997994,-18.8798216711261,-3.28464295474436));
#88168=CARTESIAN_POINT('Ctrl Pts',(20.8460383938858,-18.807145511798,-3.28026125864754));
#88169=CARTESIAN_POINT('Ctrl Pts',(20.8410597451633,-18.7345547527403,-3.27588471139231));
#88170=CARTESIAN_POINT('Ctrl Pts',(20.8323287119824,-18.6621387228754,-3.27150816413708));
#88171=CARTESIAN_POINT('Ctrl Pts',(20.8198744021611,-18.5903137016567,-3.26713161688185));
#88172=CARTESIAN_POINT('Ctrl Pts',(20.8074279906819,-18.5185342308222,-3.26275784516925));
#88173=CARTESIAN_POINT('Ctrl Pts',(20.7912630697951,-18.4473454990803,-3.25838407345666));
#88174=CARTESIAN_POINT('Ctrl Pts',(20.7714604446778,-18.3771574681937,-3.25401030174407));
#88175=CARTESIAN_POINT('Ctrl Pts',(20.7516638455656,-18.3069907957601,-3.24963786098486));
#88176=CARTESIAN_POINT('Ctrl Pts',(20.7282318707952,-18.2378246835973,-3.24526542022566));
#88177=CARTESIAN_POINT('Ctrl Pts',(20.7012957832858,-18.1700560754979,-3.24089297946646));
#88178=CARTESIAN_POINT('Ctrl Pts',(20.6743590070175,-18.102285734547,-3.23652042690342));
#88179=CARTESIAN_POINT('Ctrl Pts',(20.6439181201481,-18.0359134161341,-3.23214787434038));
#88180=CARTESIAN_POINT('Ctrl Pts',(20.610152715999,-17.9713165718493,-3.22777532177735));
#88181=CARTESIAN_POINT('Ctrl Pts',(20.5763522688392,-17.9066526865215,-3.22339823121424));
#88182=CARTESIAN_POINT('Ctrl Pts',(20.5392206395602,-17.8437683827178,-3.21902114065113));
#88183=CARTESIAN_POINT('Ctrl Pts',(20.4989832512062,-17.7830162007275,-3.21464405008802));
#88184=CARTESIAN_POINT('Ctrl Pts',(20.4587238877206,-17.7222308397152,-3.21026456903325));
#88185=CARTESIAN_POINT('Ctrl Pts',(20.4153556750976,-17.6635803070159,-3.20588508797848));
#88186=CARTESIAN_POINT('Ctrl Pts',(20.3691456171871,-17.607385627552,-3.20150560692372));
#88187=CARTESIAN_POINT('Ctrl Pts',(20.3228536522578,-17.5510913433943,-3.19711836326805));
#88188=CARTESIAN_POINT('Ctrl Pts',(20.2737101085744,-17.4972619617622,-3.19273111961239));
#88189=CARTESIAN_POINT('Ctrl Pts',(20.2220198585541,-17.4461826470157,-3.18834387595673));
#88190=CARTESIAN_POINT('Ctrl Pts',(20.1868754689112,-17.4114536344952,-3.18536097298311));
#88191=CARTESIAN_POINT('Ctrl Pts',(20.1505545743033,-17.3779951039876,-3.18237807000949));
#88192=CARTESIAN_POINT('Ctrl Pts',(20.1131612647175,-17.3458856809359,-3.17939516703586));
#88193=CARTESIAN_POINT('Ctrl Pts',(20.0581512102737,-17.2986488589,-3.17500695810766));
#88194=CARTESIAN_POINT('Ctrl Pts',(20.000604149589,-17.2541492751002,-3.17061874917945));
#88195=CARTESIAN_POINT('Ctrl Pts',(19.9408236893637,-17.212670938899,-3.16623054025124));
#88196=CARTESIAN_POINT('Ctrl Pts',(19.881131953254,-17.1712541634265,-3.16184884415272));
#88197=CARTESIAN_POINT('Ctrl Pts',(19.8192137908515,-17.1328500068488,-3.1574671480542));
#88198=CARTESIAN_POINT('Ctrl Pts',(19.7554066235781,-17.0977029608742,-3.15308545195568));
#88199=CARTESIAN_POINT('Ctrl Pts',(19.6916744348054,-17.0625972154763,-3.14870890469885));
#88200=CARTESIAN_POINT('Ctrl Pts',(19.6260580710933,-17.0307412091793,-3.14433235744203));
#88201=CARTESIAN_POINT('Ctrl Pts',(19.5589233130942,-17.0023357910877,-3.13995581018521));
#88202=CARTESIAN_POINT('Ctrl Pts',(19.4918311309837,-16.9739483872997,-3.1355820384711));
#88203=CARTESIAN_POINT('Ctrl Pts',(19.4232229083471,-16.9490074173244,-3.13120826675699));
#88204=CARTESIAN_POINT('Ctrl Pts',(19.3534870964588,-16.9276668413225,-3.12683449504287));
#88205=CARTESIAN_POINT('Ctrl Pts',(19.2837725054129,-16.9063327593298,-3.12246205428222));
#88206=CARTESIAN_POINT('Ctrl Pts',(19.2129314673181,-16.8885970372539,-3.11808961352157));
#88207=CARTESIAN_POINT('Ctrl Pts',(19.1413687992148,-16.874564161899,-3.11371717276092));
#88208=CARTESIAN_POINT('Ctrl Pts',(19.0698043012467,-16.8605309277221,-3.10934462019651));
#88209=CARTESIAN_POINT('Ctrl Pts',(18.9975186103825,-16.850200819109,-3.1049720676321));
#88210=CARTESIAN_POINT('Ctrl Pts',(18.9249263141352,-16.8436271338848,-3.10059951506769));
#88211=CARTESIAN_POINT('Ctrl Pts',(18.8522586788652,-16.8370466262422,-3.09622242450332));
#88212=CARTESIAN_POINT('Ctrl Pts',(18.7792842843309,-16.8342303693192,-3.09184533393896));
#88213=CARTESIAN_POINT('Ctrl Pts',(18.7064215783436,-16.8351796413822,-3.0874682433746));
#88214=CARTESIAN_POINT('Ctrl Pts',(18.6335190793285,-16.8361294318778,-3.08308876231864));
#88215=CARTESIAN_POINT('Ctrl Pts',(18.5607288720061,-16.8408488145897,-3.07870928126269));
#88216=CARTESIAN_POINT('Ctrl Pts',(18.4884654116526,-16.8492870462364,-3.07432980020673));
#88217=CARTESIAN_POINT('Ctrl Pts',(18.4160738648006,-16.8577402345921,-3.06994255655));
#88218=CARTESIAN_POINT('Ctrl Pts',(18.3442114053978,-16.8699253543968,-3.06555531289326));
#88219=CARTESIAN_POINT('Ctrl Pts',(18.2732828332001,-16.8857404102543,-3.06116806923653));
#88220=CARTESIAN_POINT('Ctrl Pts',(18.2250582383153,-16.896493124403,-3.05818516627583));
#88221=CARTESIAN_POINT('Ctrl Pts',(18.1772650979177,-16.9089227808441,-3.05520226331513));
#88222=CARTESIAN_POINT('Ctrl Pts',(18.1300258654966,-16.9229844148329,-3.05221936035442));
#88223=CARTESIAN_POINT('Ctrl Pts',(18.0605312740272,-16.9436707693599,-3.04783115140135));
#88224=CARTESIAN_POINT('Ctrl Pts',(17.9919650333991,-16.9679719598254,-3.04344294244828));
#88225=CARTESIAN_POINT('Ctrl Pts',(17.9247302870922,-16.9957864299187,-3.03905473349521));
#88226=CARTESIAN_POINT('Ctrl Pts',(17.8575953282951,-17.0235596187273,-3.0346730373717));
#88227=CARTESIAN_POINT('Ctrl Pts',(17.7917883829318,-17.0548355532124,-3.03029134124819));
#88228=CARTESIAN_POINT('Ctrl Pts',(17.727697669656,-17.0894628540766,-3.02590964512468));
#88229=CARTESIAN_POINT('Ctrl Pts',(17.6636822680685,-17.1240494651069,-3.02153309784279));
#88230=CARTESIAN_POINT('Ctrl Pts',(17.6013795146522,-17.1619793912541,-3.01715655056091));
#88231=CARTESIAN_POINT('Ctrl Pts',(17.5411562818509,-17.2030537846829,-3.01278000327903));
#88232=CARTESIAN_POINT('Ctrl Pts',(17.4809712417485,-17.2441021293283,-3.00840623153983));
#88233=CARTESIAN_POINT('Ctrl Pts',(17.4228635031204,-17.2882907134209,-3.00403245980062));
#88234=CARTESIAN_POINT('Ctrl Pts',(17.3671727834067,-17.3353762466239,-2.99965868806142));
#88235=CARTESIAN_POINT('Ctrl Pts',(17.3114990105664,-17.3824474515407,-2.99528624727568));
#88236=CARTESIAN_POINT('Ctrl Pts',(17.2582411645733,-17.43241354416,-2.99091380648995));
#88237=CARTESIAN_POINT('Ctrl Pts',(17.2077062220826,-17.4849906941363,-2.98654136570421));
#88238=CARTESIAN_POINT('Ctrl Pts',(17.1571699874087,-17.5375691885152,-2.98216881311475));
#88239=CARTESIAN_POINT('Ctrl Pts',(17.1093571273004,-17.5927585236412,-2.9777962605253));
#88240=CARTESIAN_POINT('Ctrl Pts',(17.0645368651535,-17.650238946124,-2.97342370793584));
#88241=CARTESIAN_POINT('Ctrl Pts',(17.0196700868509,-17.7077790239535,-2.96904661734668));
#88242=CARTESIAN_POINT('Ctrl Pts',(16.977802404763,-17.7676145553151,-2.96466952675751));
#88243=CARTESIAN_POINT('Ctrl Pts',(16.9391613915751,-17.8293943837182,-2.96029243616834));
#88244=CARTESIAN_POINT('Ctrl Pts',(16.9004992750969,-17.8912079523768,-2.95591295508767));
#88245=CARTESIAN_POINT('Ctrl Pts',(16.8650675705235,-17.9549675102763,-2.951533474007));
#88246=CARTESIAN_POINT('Ctrl Pts',(16.833047947568,-18.0202970997391,-2.94715399292634));
#88247=CARTESIAN_POINT('Ctrl Pts',(16.8009715700491,-18.0857424854538,-2.94276674924532));
#88248=CARTESIAN_POINT('Ctrl Pts',(16.7723195413291,-18.1527630160747,-2.93837950556431));
#88249=CARTESIAN_POINT('Ctrl Pts',(16.7472252098534,-18.2209631108913,-2.93399226188329));
#88250=CARTESIAN_POINT('Ctrl Pts',(16.7301634837495,-18.2673326003173,-2.93100935914652));
#88251=CARTESIAN_POINT('Ctrl Pts',(16.7147453386169,-18.3142470017708,-2.92802645640976));
#88252=CARTESIAN_POINT('Ctrl Pts',(16.7009992479662,-18.3615790127122,-2.92504355367299));
#88253=CARTESIAN_POINT('Ctrl Pts',(16.6758066766596,-18.4483247712722,-2.91957676374658));
#88254=CARTESIAN_POINT('Ctrl Pts',(16.6561521069762,-18.5367464915003,-2.91410997382017));
#88255=CARTESIAN_POINT('Ctrl Pts',(16.642218086188,-18.6262126075965,-2.90864318389376));
#88256=CARTESIAN_POINT('Ctrl Pts',(16.6285119268969,-18.714215694215,-2.90326579177692));
#88257=CARTESIAN_POINT('Ctrl Pts',(16.6203407792491,-18.8032293912184,-2.89788839966009));
#88258=CARTESIAN_POINT('Ctrl Pts',(16.6178326248384,-18.8926313188492,-2.89251100754326));
#88259=CARTESIAN_POINT('Ctrl Pts',(16.6172955000024,-18.9117768688659,-2.89135943136967));
#88260=CARTESIAN_POINT('Ctrl Pts',(16.6170179137274,-18.9309401417671,-2.89020785519609));
#88261=CARTESIAN_POINT('Ctrl Pts',(16.6170008393112,-18.9501148891278,-2.8890562790225));
#88262=CARTESIAN_POINT('Ctrl Pts',(16.618038032075,-18.9501158127103,-2.8890562790225));
#88263=CARTESIAN_POINT('Ctrl Pts',(16.6201501825404,-19.1969463155021,-2.87422525894902));
#88264=CARTESIAN_POINT('Ctrl Pts',(16.664522062029,-19.4444420314544,-2.85939423887553));
#88265=CARTESIAN_POINT('Ctrl Pts',(16.7477770216415,-19.6772709618372,-2.84456321880205));
#88266=CARTESIAN_POINT('Origin',(18.734,-18.952,0.));
#88267=CARTESIAN_POINT('',(16.7454194493934,-19.6781104556121,-2.04625066941376));
#88268=CARTESIAN_POINT('',(16.7454194499845,-19.6781104572309,-2.26547385582022));
#88269=CARTESIAN_POINT('',(16.7454194499637,-19.6781104571739,0.));
#88270=CARTESIAN_POINT('',(16.617000743883,-18.9537747113038,-2.31031846929929));
#88271=CARTESIAN_POINT('Ctrl Pts',(16.7454194499845,-19.6781104572309,-2.26547385582022));
#88272=CARTESIAN_POINT('Ctrl Pts',(16.7104732804469,-19.5824042566824,-2.27104574889238));
#88273=CARTESIAN_POINT('Ctrl Pts',(16.6824859377261,-19.4843109672804,-2.27670318400123));
#88274=CARTESIAN_POINT('Ctrl Pts',(16.6596908892846,-19.3751129893312,-2.28331203840856));
#88275=CARTESIAN_POINT('Ctrl Pts',(16.6577760537803,-19.3656145616665,-2.2838894546805));
#88276=CARTESIAN_POINT('Ctrl Pts',(16.6550449338362,-19.3515699728654,-2.28474744876694));
#88277=CARTESIAN_POINT('Ctrl Pts',(16.6541781832451,-19.347033593467,-2.28502522690602));
#88278=CARTESIAN_POINT('Ctrl Pts',(16.652666747724,-19.3389802036193,-2.28551956976332));
#88279=CARTESIAN_POINT('Ctrl Pts',(16.6520161213478,-19.3354643579864,-2.28573579285723));
#88280=CARTESIAN_POINT('Ctrl Pts',(16.6506410990766,-19.3279273650159,-2.28620020863802));
#88281=CARTESIAN_POINT('Ctrl Pts',(16.6499194471366,-19.3239058245693,-2.28644854782864));
#88282=CARTESIAN_POINT('Ctrl Pts',(16.6484623845843,-19.3156486440134,-2.28695951762119));
#88283=CARTESIAN_POINT('Ctrl Pts',(16.6477282255922,-19.311412804693,-2.28722221639482));
#88284=CARTESIAN_POINT('Ctrl Pts',(16.6459029140947,-19.30068734686,-2.28788879786091));
#88285=CARTESIAN_POINT('Ctrl Pts',(16.644829118727,-19.2941948747727,-2.28829360523636));
#88286=CARTESIAN_POINT('Ctrl Pts',(16.6260482815475,-19.1772563681001,-2.29560690850301));
#88287=CARTESIAN_POINT('Ctrl Pts',(16.6170944875345,-19.0655986682839,-2.30293671225118));
#88288=CARTESIAN_POINT('Ctrl Pts',(16.617000743883,-18.9537747113038,-2.31031846929929));
#88289=CARTESIAN_POINT('Ctrl Pts',(16.6170007453241,-18.9537764294638,-2.31031835587959));
#88290=CARTESIAN_POINT('Ctrl Pts',(16.6169157267001,-18.8524583825956,-2.3170065931235));
#88291=CARTESIAN_POINT('Ctrl Pts',(16.624104387429,-18.751255842761,-2.32371995685458));
#88292=CARTESIAN_POINT('Ctrl Pts',(16.6510544988285,-18.5636665537717,-2.33599025543251));
#88293=CARTESIAN_POINT('Ctrl Pts',(16.6690366508714,-18.4772425906475,-2.34157367536228));
#88294=CARTESIAN_POINT('Ctrl Pts',(16.6977848563535,-18.3723986625979,-2.34824549634076));
#88295=CARTESIAN_POINT('Ctrl Pts',(16.7034969582071,-18.3526943473505,-2.34949515434532));
#88296=CARTESIAN_POINT('Ctrl Pts',(16.7120848616524,-18.3246032652549,-2.35127114804834));
#88297=CARTESIAN_POINT('Ctrl Pts',(16.7147281849505,-18.3161471631551,-2.35180504107459));
#88298=CARTESIAN_POINT('Ctrl Pts',(16.7194026267417,-18.3015165893118,-2.35272758592687));
#88299=CARTESIAN_POINT('Ctrl Pts',(16.7214092263582,-18.2953344662358,-2.35311703688876));
#88300=CARTESIAN_POINT('Ctrl Pts',(16.7253221590219,-18.2834655559935,-2.35386406073909));
#88301=CARTESIAN_POINT('Ctrl Pts',(16.7272242478572,-18.2777774451925,-2.35422176907291));
#88302=CARTESIAN_POINT('Ctrl Pts',(16.7322704288395,-18.2628976165899,-2.35515677610282));
#88303=CARTESIAN_POINT('Ctrl Pts',(16.7354536843469,-18.2537192542765,-2.35573277519751));
#88304=CARTESIAN_POINT('Ctrl Pts',(16.7467207700364,-18.2219408543608,-2.35772474837877));
#88305=CARTESIAN_POINT('Ctrl Pts',(16.7551258655886,-18.1994560987812,-2.35913005312993));
#88306=CARTESIAN_POINT('Ctrl Pts',(16.8192013078531,-18.0365482671872,-2.36929206489179));
#88307=CARTESIAN_POINT('Ctrl Pts',(16.8893770781872,-17.9022957692239,-2.37751640320179));
#88308=CARTESIAN_POINT('Ctrl Pts',(17.010444033627,-17.7209310046249,-2.3893581083965));
#88309=CARTESIAN_POINT('Ctrl Pts',(17.0502564563995,-17.6670162703443,-2.39299175397592));
#88310=CARTESIAN_POINT('Ctrl Pts',(17.1266260981131,-17.5732510489217,-2.39967845901954));
#88311=CARTESIAN_POINT('Ctrl Pts',(17.162280234728,-17.5327411408619,-2.40270478382399));
#88312=CARTESIAN_POINT('Ctrl Pts',(17.2186822880118,-17.4733920444582,-2.40743003576606));
#88313=CARTESIAN_POINT('Ctrl Pts',(17.2383226321031,-17.4535280131053,-2.40906498891257));
#88314=CARTESIAN_POINT('Ctrl Pts',(17.2632324301722,-17.429312199152,-2.41113481132057));
#88315=CARTESIAN_POINT('Ctrl Pts',(17.2681385497757,-17.4245885985822,-2.41154229695243));
#88316=CARTESIAN_POINT('Ctrl Pts',(17.2760238299547,-17.417069650961,-2.4121971076798));
#88317=CARTESIAN_POINT('Ctrl Pts',(17.2789884850262,-17.4142590662059,-2.41244327356044));
#88318=CARTESIAN_POINT('Ctrl Pts',(17.2845632967386,-17.4090045271771,-2.41290616490901));
#88319=CARTESIAN_POINT('Ctrl Pts',(17.2871715164566,-17.406558598833,-2.4131227341679));
#88320=CARTESIAN_POINT('Ctrl Pts',(17.2931635024018,-17.4009679156958,-2.41362026277763));
#88321=CARTESIAN_POINT('Ctrl Pts',(17.2965513637841,-17.3978276296821,-2.4139015569804));
#88322=CARTESIAN_POINT('Ctrl Pts',(17.3070809758866,-17.3881313723651,-2.41477572904382));
#88323=CARTESIAN_POINT('Ctrl Pts',(17.3142573847721,-17.3816134602653,-2.4153713724465));
#88324=CARTESIAN_POINT('Ctrl Pts',(17.3958754273366,-17.3085012945656,-2.42214147294141));
#88325=CARTESIAN_POINT('Ctrl Pts',(17.4748875437639,-17.2472136638242,-2.42865076829811));
#88326=CARTESIAN_POINT('Ctrl Pts',(17.6997491507202,-17.0969771327951,-2.44646869862621));
#88327=CARTESIAN_POINT('Ctrl Pts',(17.8525403061836,-17.0196875560976,-2.45779497513617));
#88328=CARTESIAN_POINT('Ctrl Pts',(18.0405779362481,-16.9515707138203,-2.47032890480205));
#88329=CARTESIAN_POINT('Ctrl Pts',(18.0683963355061,-16.9421434421884,-2.47215154346896));
#88330=CARTESIAN_POINT('Ctrl Pts',(18.1167124537869,-16.9268830388013,-2.47526360868176));
#88331=CARTESIAN_POINT('Ctrl Pts',(18.1371181024035,-16.9207750805008,-2.47656174562872));
#88332=CARTESIAN_POINT('Ctrl Pts',(18.1662673119798,-16.9125271544833,-2.47839376932748));
#88333=CARTESIAN_POINT('Ctrl Pts',(18.1749371893979,-16.9101335326837,-2.47893588316393));
#88334=CARTESIAN_POINT('Ctrl Pts',(18.1899213291353,-16.9060992312121,-2.47986809349407));
#88335=CARTESIAN_POINT('Ctrl Pts',(18.1962283538843,-16.9044323664579,-2.48025903543764));
#88336=CARTESIAN_POINT('Ctrl Pts',(18.2083198987657,-16.9012964504983,-2.48100581831021));
#88337=CARTESIAN_POINT('Ctrl Pts',(18.2141031140155,-16.8998226573126,-2.48136180949962));
#88338=CARTESIAN_POINT('Ctrl Pts',(18.2291591998643,-16.8960534979491,-2.48228556538595));
#88339=CARTESIAN_POINT('Ctrl Pts',(18.2384415780601,-16.8937963881657,-2.48285209172705));
#88340=CARTESIAN_POINT('Ctrl Pts',(18.2701539036314,-16.8863121704246,-2.48477764924978));
#88341=CARTESIAN_POINT('Ctrl Pts',(18.2926542168509,-16.8813881649859,-2.48612695359053));
#88342=CARTESIAN_POINT('Ctrl Pts',(18.4867167624519,-16.8422263379409,-2.49763049943239));
#88343=CARTESIAN_POINT('Ctrl Pts',(18.6618284568133,-16.8290087383454,-2.50703923594699));
#88344=CARTESIAN_POINT('Ctrl Pts',(18.9238618204368,-16.8417211768299,-2.52131227346742));
#88345=CARTESIAN_POINT('Ctrl Pts',(19.0107864267335,-16.8513546041382,-2.5260947730487));
#88346=CARTESIAN_POINT('Ctrl Pts',(19.1342164402318,-16.8728286295504,-2.53324710796108));
#88347=CARTESIAN_POINT('Ctrl Pts',(19.1713895143418,-16.8803299496605,-2.53544951018984));
#88348=CARTESIAN_POINT('Ctrl Pts',(19.2157229109256,-16.8905225080335,-2.5381560102116));
#88349=CARTESIAN_POINT('Ctrl Pts',(19.2230980911231,-16.8922598547094,-2.53860893189092));
#88350=CARTESIAN_POINT('Ctrl Pts',(19.234530439768,-16.8950177978229,-2.53931539356148));
#88351=CARTESIAN_POINT('Ctrl Pts',(19.2385942632114,-16.8960109119826,-2.53956737935247));
#88352=CARTESIAN_POINT('Ctrl Pts',(19.2461143690509,-16.8978723085235,-2.54003532144812));
#88353=CARTESIAN_POINT('Ctrl Pts',(19.2495714127354,-16.8987372750501,-2.54025108545263));
#88354=CARTESIAN_POINT('Ctrl Pts',(19.2573681691612,-16.9007089876509,-2.54073916213289));
#88355=CARTESIAN_POINT('Ctrl Pts',(19.2617065382762,-16.901820772117,-2.54101176133799));
#88356=CARTESIAN_POINT('Ctrl Pts',(19.2744608351391,-16.9051324533573,-2.54181609981238));
#88357=CARTESIAN_POINT('Ctrl Pts',(19.2828666506179,-16.9073704341119,-2.54234996337193));
#88358=CARTESIAN_POINT('Ctrl Pts',(19.3423525785472,-16.9236013393259,-2.54615349330763));
#88359=CARTESIAN_POINT('Ctrl Pts',(19.3929012966376,-16.939453838755,-2.54951885175871));
#88360=CARTESIAN_POINT('Ctrl Pts',(19.4568597127052,-16.9621795200576,-2.55390448736739));
#88361=CARTESIAN_POINT('Ctrl Pts',(19.4708683067114,-16.9673245126588,-2.55487308977862));
#88362=CARTESIAN_POINT('Ctrl Pts',(19.6170531287681,-17.0227754547697,-2.56505777558374));
#88363=CARTESIAN_POINT('Ctrl Pts',(19.7439283666313,-17.086058305033,-2.57452807062539));
#88364=CARTESIAN_POINT('Ctrl Pts',(19.9496497124028,-17.2158410060306,-2.59031032917732));
#88365=CARTESIAN_POINT('Ctrl Pts',(20.0317277331629,-17.2763030431253,-2.59675072266805));
#88366=CARTESIAN_POINT('Ctrl Pts',(20.1203794467244,-17.3520439602973,-2.60386108689854));
#88367=CARTESIAN_POINT('Ctrl Pts',(20.1315122679663,-17.3617588932709,-2.60475721462031));
#88368=CARTESIAN_POINT('Ctrl Pts',(20.1483371791712,-17.3767541175907,-2.60611671649479));
#88369=CARTESIAN_POINT('Ctrl Pts',(20.1541032746538,-17.3819503389213,-2.60658358309978));
#88370=CARTESIAN_POINT('Ctrl Pts',(20.1645426076581,-17.3914624930856,-2.60743061977818));
#88371=CARTESIAN_POINT('Ctrl Pts',(20.169225198764,-17.3957679822686,-2.60781122426496));
#88372=CARTESIAN_POINT('Ctrl Pts',(20.1792933467162,-17.4051094076467,-2.60863104962916));
#88373=CARTESIAN_POINT('Ctrl Pts',(20.1846721564752,-17.4101525174941,-2.60906995727571));
#88374=CARTESIAN_POINT('Ctrl Pts',(20.1991874877773,-17.4239051232286,-2.61025700308935));
#88375=CARTESIAN_POINT('Ctrl Pts',(20.2082727311446,-17.4326684853727,-2.61100280888896));
#88376=CARTESIAN_POINT('Ctrl Pts',(20.2521097091861,-17.4757158377018,-2.61461612905962));
#88377=CARTESIAN_POINT('Ctrl Pts',(20.2857484979255,-17.5111151482182,-2.61743409475524));
#88378=CARTESIAN_POINT('Ctrl Pts',(20.3451760363231,-17.5781505238545,-2.62252471944323));
#88379=CARTESIAN_POINT('Ctrl Pts',(20.3713310545648,-17.6094286367836,-2.62480961838324));
#88380=CARTESIAN_POINT('Ctrl Pts',(20.4697251199958,-17.7342510388125,-2.63362949005832));
#88381=CARTESIAN_POINT('Ctrl Pts',(20.5349825190024,-17.833019847798,-2.63996753077614));
#88382=CARTESIAN_POINT('Ctrl Pts',(20.6274746363598,-18.0022525173367,-2.65050223644797));
#88383=CARTESIAN_POINT('Ctrl Pts',(20.6597957065887,-18.0696306559827,-2.6546248085828));
#88384=CARTESIAN_POINT('Ctrl Pts',(20.7017512318337,-18.1704401716056,-2.66088070154777));
#88385=CARTESIAN_POINT('Ctrl Pts',(20.7142329780273,-18.2026284504811,-2.66289096454807));
#88386=CARTESIAN_POINT('Ctrl Pts',(20.7284180183301,-18.2420421694957,-2.66538431436342));
#88387=CARTESIAN_POINT('Ctrl Pts',(20.7308783061947,-18.2489919064815,-2.66582514823603));
#88388=CARTESIAN_POINT('Ctrl Pts',(20.734663004152,-18.259862966046,-2.66651677603205));
#88389=CARTESIAN_POINT('Ctrl Pts',(20.7360123274733,-18.2637756398353,-2.6667661188903));
#88390=CARTESIAN_POINT('Ctrl Pts',(20.7385035381253,-18.2710688013267,-2.66723170512251));
#88391=CARTESIAN_POINT('Ctrl Pts',(20.7396483557959,-18.2744482278453,-2.66744777238327));
#88392=CARTESIAN_POINT('Ctrl Pts',(20.7422300765555,-18.2821331761196,-2.66793985755675));
#88393=CARTESIAN_POINT('Ctrl Pts',(20.7436616732755,-18.2864404157414,-2.66821618275783));
#88394=CARTESIAN_POINT('Ctrl Pts',(20.7478845501271,-18.2992836196729,-2.66904160543179));
#88395=CARTESIAN_POINT('Ctrl Pts',(20.750635335215,-18.307832651712,-2.66959299347377));
#88396=CARTESIAN_POINT('Ctrl Pts',(20.771487346728,-18.3740803590518,-2.67387940629834));
#88397=CARTESIAN_POINT('Ctrl Pts',(20.7871615666049,-18.4325079965425,-2.67773895612883));
#88398=CARTESIAN_POINT('Ctrl Pts',(20.8133953508008,-18.5502268830383,-2.68556754238047));
#88399=CARTESIAN_POINT('Ctrl Pts',(20.823969939628,-18.6094626852835,-2.68953238882852));
#88400=CARTESIAN_POINT('Ctrl Pts',(20.8465536991121,-18.7769254187073,-2.70069588184445));
#88401=CARTESIAN_POINT('Ctrl Pts',(20.8527612528954,-18.8857544456839,-2.70788913114571));
#88402=CARTESIAN_POINT('Ctrl Pts',(20.8490664369905,-19.0693984680566,-2.71968940138976));
#88403=CARTESIAN_POINT('Ctrl Pts',(20.8435955456403,-19.1440864297013,-2.72439685678408));
#88404=CARTESIAN_POINT('Ctrl Pts',(20.8318169690626,-19.2369660491584,-2.73013210059552));
#88405=CARTESIAN_POINT('Ctrl Pts',(20.8292064467372,-19.2555649289488,-2.73127472609475));
#88406=CARTESIAN_POINT('Ctrl Pts',(20.8250478441223,-19.2825767731772,-2.73292612749323));
#88407=CARTESIAN_POINT('Ctrl Pts',(20.8236957881941,-19.2910185917114,-2.73344107780867));
#88408=CARTESIAN_POINT('Ctrl Pts',(20.8212342700186,-19.3058130639097,-2.7343415863058));
#88409=CARTESIAN_POINT('Ctrl Pts',(20.8201468576687,-19.312169226613,-2.73472783867462));
#88410=CARTESIAN_POINT('Ctrl Pts',(20.8179779285443,-19.3245076488993,-2.73547642559675));
#88411=CARTESIAN_POINT('Ctrl Pts',(20.8168996538134,-19.3304904073792,-2.73583885903512));
#88412=CARTESIAN_POINT('Ctrl Pts',(20.8142586323714,-19.3447908430385,-2.73670390423305));
#88413=CARTESIAN_POINT('Ctrl Pts',(20.8126717417312,-19.3531039980098,-2.73720574370037));
#88414=CARTESIAN_POINT('Ctrl Pts',(20.8067546261789,-19.3831231257994,-2.73901436199857));
#88415=CARTESIAN_POINT('Ctrl Pts',(20.8021338201563,-19.4047708541332,-2.74031188241666));
#88416=CARTESIAN_POINT('Ctrl Pts',(20.755647546784,-19.6069649012208,-2.75237798096232));
#88417=CARTESIAN_POINT('Ctrl Pts',(20.6905855127162,-19.7813473298862,-2.76229272251722));
#88418=CARTESIAN_POINT('Ctrl Pts',(20.5659711476454,-20.0159642293777,-2.77677404847788));
#88419=CARTESIAN_POINT('Ctrl Pts',(20.524298620227,-20.0846813329277,-2.7811898915694));
#88420=CARTESIAN_POINT('Ctrl Pts',(20.4583989091041,-20.1805921910746,-2.78784597860492));
#88421=CARTESIAN_POINT('Ctrl Pts',(20.4372145872169,-20.2097957265714,-2.78994422700567));
#88422=CARTESIAN_POINT('Ctrl Pts',(20.4107574033016,-20.244373551044,-2.79253523742792));
#88423=CARTESIAN_POINT('Ctrl Pts',(20.4061874580466,-20.2502811276242,-2.79298177026394));
#88424=CARTESIAN_POINT('Ctrl Pts',(20.3990237391862,-20.2594411087297,-2.79368039379265));
#88425=CARTESIAN_POINT('Ctrl Pts',(20.3964514258274,-20.2627103268574,-2.79393098518313));
#88426=CARTESIAN_POINT('Ctrl Pts',(20.3916562811557,-20.2687677733069,-2.79439767245135));
#88427=CARTESIAN_POINT('Ctrl Pts',(20.3894360349361,-20.2715579748176,-2.79461358453165));
#88428=CARTESIAN_POINT('Ctrl Pts',(20.3843918206881,-20.277864312852,-2.79510372197686));
#88429=CARTESIAN_POINT('Ctrl Pts',(20.3815636745789,-20.2813770252365,-2.79537824459905));
#88430=CARTESIAN_POINT('Ctrl Pts',(20.3742331264094,-20.2904226447702,-2.79608901776612));
#88431=CARTESIAN_POINT('Ctrl Pts',(20.3697139862928,-20.2959418278869,-2.7965264340528));
#88432=CARTESIAN_POINT('Ctrl Pts',(20.3418038920467,-20.3296788566898,-2.79922269906642));
#88433=CARTESIAN_POINT('Ctrl Pts',(20.3177127680746,-20.3573063305051,-2.80152770030752));
#88434=CARTESIAN_POINT('Ctrl Pts',(20.1775005399055,-20.5099144196942,-2.8147531387914));
#88435=CARTESIAN_POINT('Ctrl Pts',(20.047323332482,-20.6211243468025,-2.82626428826224));
#88436=CARTESIAN_POINT('Ctrl Pts',(19.8257930265195,-20.7682503569405,-2.84354607192485));
#88437=CARTESIAN_POINT('Ctrl Pts',(19.7428987052606,-20.8155731859445,-2.84960289451251));
#88438=CARTESIAN_POINT('Ctrl Pts',(19.6378403464578,-20.8664761590398,-2.85677370751244));
#88439=CARTESIAN_POINT('Ctrl Pts',(19.6184542690078,-20.8755090418604,-2.85807722426939));
#88440=CARTESIAN_POINT('Ctrl Pts',(19.5907115234959,-20.8879275614428,-2.85991545080504));
#88441=CARTESIAN_POINT('Ctrl Pts',(19.5824654666089,-20.8915557515932,-2.86045846365643));
#88442=CARTESIAN_POINT('Ctrl Pts',(19.5682062357659,-20.8977213435956,-2.86139173415881));
#88443=CARTESIAN_POINT('Ctrl Pts',(19.5622040752749,-20.9002837580529,-2.86178284235533));
#88444=CARTESIAN_POINT('Ctrl Pts',(19.5506934294096,-20.9051350241594,-2.86252961278044));
#88445=CARTESIAN_POINT('Ctrl Pts',(19.5451869406504,-20.9074284258645,-2.86288542685636));
#88446=CARTESIAN_POINT('Ctrl Pts',(19.5308526032992,-20.9133275756213,-2.86380801029628));
#88447=CARTESIAN_POINT('Ctrl Pts',(19.522009891795,-20.9168970317126,-2.86437354764334));
#88448=CARTESIAN_POINT('Ctrl Pts',(19.491824715731,-20.9288450588684,-2.86629208835762));
#88449=CARTESIAN_POINT('Ctrl Pts',(19.4703699202056,-20.9369367968764,-2.86763546233721));
#88450=CARTESIAN_POINT('Ctrl Pts',(19.2828170677453,-21.0042132700977,-2.87921454337805));
#88451=CARTESIAN_POINT('Ctrl Pts',(19.1100620526455,-21.0427805890613,-2.88869091057756));
#88452=CARTESIAN_POINT('Ctrl Pts',(18.8484861431891,-21.0676675513043,-2.90298972081201));
#88453=CARTESIAN_POINT('Ctrl Pts',(18.7620473751143,-21.0705767034938,-2.90772225827461));
#88454=CARTESIAN_POINT('Ctrl Pts',(18.6380215811988,-21.0671587206841,-2.91480722856474));
#88455=CARTESIAN_POINT('Ctrl Pts',(18.6003996697387,-21.065115904893,-2.91699580783972));
#88456=CARTESIAN_POINT('Ctrl Pts',(18.5553166277762,-21.0614592798462,-2.91968698669883));
#88457=CARTESIAN_POINT('Ctrl Pts',(18.5477817190871,-21.0608074707712,-2.92013908174524));
#88458=CARTESIAN_POINT('Ctrl Pts',(18.5360877334676,-21.0597327180037,-2.92084452954647));
#88459=CARTESIAN_POINT('Ctrl Pts',(18.5319260564627,-21.0593377983695,-2.92109633525314));
#88460=CARTESIAN_POINT('Ctrl Pts',(18.5242186248803,-21.0585833656314,-2.92156411387037));
#88461=CARTESIAN_POINT('Ctrl Pts',(18.5206725982112,-21.0582272243907,-2.92177989557451));
#88462=CARTESIAN_POINT('Ctrl Pts',(18.5126685294896,-21.0574029242214,-2.92226823193328));
#88463=CARTESIAN_POINT('Ctrl Pts',(18.5082110906084,-21.0569295619329,-2.9225410744761));
#88464=CARTESIAN_POINT('Ctrl Pts',(18.4950899266296,-21.0554939893562,-2.92334678203535));
#88465=CARTESIAN_POINT('Ctrl Pts',(18.486430725204,-21.054492433896,-2.9238817819525));
#88466=CARTESIAN_POINT('Ctrl Pts',(18.4248693935503,-21.0469864481336,-2.92770744946584));
#88467=CARTESIAN_POINT('Ctrl Pts',(18.3722277688613,-21.0385401430755,-2.93109502138744));
#88468=CARTESIAN_POINT('Ctrl Pts',(18.3023662881824,-21.0246078762941,-2.93569887498028));
#88469=CARTESIAN_POINT('Ctrl Pts',(18.2848122311734,-21.0208744265362,-2.93686496398954));
#88470=CARTESIAN_POINT('Ctrl Pts',(18.2202645661322,-21.0062860186564,-2.94118251760858));
#88471=CARTESIAN_POINT('Ctrl Pts',(18.1735992369101,-20.9940494347733,-2.94436203543676));
#88472=CARTESIAN_POINT('Ctrl Pts',(18.0226006314629,-20.9488885436691,-2.95477314597037));
#88473=CARTESIAN_POINT('Ctrl Pts',(17.9203858758801,-20.9094699078853,-2.96200572004032));
#88474=CARTESIAN_POINT('Ctrl Pts',(17.753380782476,-20.8297119156859,-2.97390170928805));
#88475=CARTESIAN_POINT('Ctrl Pts',(17.6868835548687,-20.7934574222726,-2.97866451213787));
#88476=CARTESIAN_POINT('Ctrl Pts',(17.6063837261286,-20.7437945036205,-2.98445946774088));
#88477=CARTESIAN_POINT('Ctrl Pts',(17.5904362791863,-20.7336587936744,-2.98560916449256));
#88478=CARTESIAN_POINT('Ctrl Pts',(17.567455414304,-20.7186171570415,-2.98726883608506));
#88479=CARTESIAN_POINT('Ctrl Pts',(17.5603130665701,-20.7138800854883,-2.98778507263282));
#88480=CARTESIAN_POINT('Ctrl Pts',(17.5478447349675,-20.705501158092,-2.98868706526776));
#88481=CARTESIAN_POINT('Ctrl Pts',(17.5425063035609,-20.701878109175,-2.98907352259808));
#88482=CARTESIAN_POINT('Ctrl Pts',(17.5321751850707,-20.6947974621759,-2.98982195238016));
#88483=CARTESIAN_POINT('Ctrl Pts',(17.5271806548056,-20.6913426773335,-2.99018402632301));
#88484=CARTESIAN_POINT('Ctrl Pts',(17.5152808115313,-20.6830354609618,-2.99104733259559));
#88485=CARTESIAN_POINT('Ctrl Pts',(17.5083894795699,-20.678163110136,-2.99154779975037));
#88486=CARTESIAN_POINT('Ctrl Pts',(17.4836528536416,-20.6604508542082,-2.99334629434098));
#88487=CARTESIAN_POINT('Ctrl Pts',(17.4659782969115,-20.6473740948702,-2.99463520021195));
#88488=CARTESIAN_POINT('Ctrl Pts',(17.3000934833205,-20.520596329793,-3.00677957041232));
#88489=CARTESIAN_POINT('Ctrl Pts',(17.1673452117098,-20.3880296027907,-3.01676512262662));
#88490=CARTESIAN_POINT('Ctrl Pts',(17.0054419400624,-20.1767742720821,-3.03127849722977));
#88491=CARTESIAN_POINT('Ctrl Pts',(16.9607582404278,-20.1111361796354,-3.03564442048094));
#88492=CARTESIAN_POINT('Ctrl Pts',(16.9014072608096,-20.0124600760732,-3.04223259877066));
#88493=CARTESIAN_POINT('Ctrl Pts',(16.8837303625087,-19.9813073624741,-3.04431617115616));
#88494=CARTESIAN_POINT('Ctrl Pts',(16.8633406663623,-19.9431499418684,-3.0468908986835));
#88495=CARTESIAN_POINT('Ctrl Pts',(16.8598628495763,-19.9365580162922,-3.04733650074735));
#88496=CARTESIAN_POINT('Ctrl Pts',(16.8544998906645,-19.92626157436,-3.04803398195452));
#88497=CARTESIAN_POINT('Ctrl Pts',(16.8525906881932,-19.9225695632107,-3.04828436972068));
#88498=CARTESIAN_POINT('Ctrl Pts',(16.8490636424379,-19.9156994581905,-3.04875087592216));
#88499=CARTESIAN_POINT('Ctrl Pts',(16.8474429522759,-19.9125228903311,-3.04896681180847));
#88500=CARTESIAN_POINT('Ctrl Pts',(16.8437887971301,-19.9053157864152,-3.04945726008974));
#88501=CARTESIAN_POINT('Ctrl Pts',(16.8417602037729,-19.9012828518333,-3.04973207134966));
#88502=CARTESIAN_POINT('Ctrl Pts',(16.8357860126926,-19.889310652084,-3.05054889576093));
#88503=CARTESIAN_POINT('Ctrl Pts',(16.8318774283855,-19.8813531709565,-3.05109313093092));
#88504=CARTESIAN_POINT('Ctrl Pts',(16.8031430628197,-19.8219122699709,-3.05516697329311));
#88505=CARTESIAN_POINT('Ctrl Pts',(16.7803635901166,-19.7694713478007,-3.05880792375393));
#88506=CARTESIAN_POINT('Ctrl Pts',(16.7548404842599,-19.7035321072633,-3.06338856020301));
#88507=CARTESIAN_POINT('Ctrl Pts',(16.750068293043,-19.6908421265627,-3.06427024202607));
#88508=CARTESIAN_POINT('Ctrl Pts',(16.7454194663415,-19.6781105020273,-3.06515442754877));
#88509=CARTESIAN_POINT('',(16.6200858902598,-18.9528284544197,-2.08900426920411));
#88510=CARTESIAN_POINT('Ctrl Pts',(16.7477770216415,-19.6772709618372,-2.84456321880205));
#88511=CARTESIAN_POINT('Ctrl Pts',(16.835153111315,-19.9216249510097,-2.82899806153188));
#88512=CARTESIAN_POINT('Ctrl Pts',(17.3199691704515,-20.7713282302527,-2.77104096870124));
#88513=CARTESIAN_POINT('Ctrl Pts',(19.0938031538723,-21.4292709570805,-2.67069194031012));
#88514=CARTESIAN_POINT('Ctrl Pts',(21.0117474660562,-19.9903622879567,-2.54351613362868));
#88515=CARTESIAN_POINT('Ctrl Pts',(20.8399998530167,-17.5988206232279,-2.41634032694726));
#88516=CARTESIAN_POINT('Ctrl Pts',(18.7361280842055,-16.4487371345171,-2.28916452026581));
#88517=CARTESIAN_POINT('Ctrl Pts',(16.9296978913047,-17.4322383584724,-2.18006983762423));
#88518=CARTESIAN_POINT('Ctrl Pts',(16.621605651229,-18.5471996814609,-2.11336709054313));
#88519=CARTESIAN_POINT('Ctrl Pts',(16.6201761380985,-18.9528314139021,-2.0890562790225));
#88520=CARTESIAN_POINT('Ctrl Pts',(16.6170001249202,-18.9527272634281,-2.08722594301759));
#88521=CARTESIAN_POINT('Ctrl Pts',(16.6170670028625,-19.1474030713124,-2.07601658058626));
#88522=CARTESIAN_POINT('Ctrl Pts',(16.6439835862141,-19.3411372612755,-2.06573526128042));
#88523=CARTESIAN_POINT('Ctrl Pts',(16.7112838360481,-19.5789443055377,-2.05215235255094));
#88524=CARTESIAN_POINT('Ctrl Pts',(16.7274347388846,-19.6288561785945,-2.04923738357229));
#88525=CARTESIAN_POINT('Ctrl Pts',(16.7454194493934,-19.6781104556121,-2.04625066941376));
#88526=CARTESIAN_POINT('Origin',(18.734,-18.952,0.));
#88527=CARTESIAN_POINT('',(16.7454193881274,-19.6781102878245,-1.24458621709266));
#88528=CARTESIAN_POINT('',(16.7454194501222,-19.6781104576079,-1.46829794770746));
#88529=CARTESIAN_POINT('',(16.7454194499637,-19.6781104571739,0.));
#88530=CARTESIAN_POINT('Ctrl Pts',(16.7454194501221,-19.6781104576079,-1.46829794770746));
#88531=CARTESIAN_POINT('Ctrl Pts',(16.6959068596802,-19.5425115644984,-1.47674752143155));
#88532=CARTESIAN_POINT('Ctrl Pts',(16.660389350048,-19.4021955419597,-1.4846915217345));
#88533=CARTESIAN_POINT('Ctrl Pts',(16.6244283767819,-19.1571126854122,-1.49816091871139));
#88534=CARTESIAN_POINT('Ctrl Pts',(16.6169334231157,-19.0539337982303,-1.50372411700594));
#88535=CARTESIAN_POINT('Ctrl Pts',(16.6170394069824,-18.8905719711407,-1.51286251429508));
#88536=CARTESIAN_POINT('Ctrl Pts',(16.6196337799717,-18.830551892442,-1.51629224317771));
#88537=CARTESIAN_POINT('Ctrl Pts',(16.6255428334935,-18.761795416016,-1.52038548468644));
#88538=CARTESIAN_POINT('Ctrl Pts',(16.6263673814007,-18.7528665137208,-1.52092024802311));
#88539=CARTESIAN_POINT('Ctrl Pts',(16.6276944044936,-18.7394292741622,-1.5217302094326));
#88540=CARTESIAN_POINT('Ctrl Pts',(16.6281546985465,-18.7349167426731,-1.52200309516185));
#88541=CARTESIAN_POINT('Ctrl Pts',(16.6290029479853,-18.7268575103288,-1.52249209211128));
#88542=CARTESIAN_POINT('Ctrl Pts',(16.6293853699247,-18.7233102795055,-1.52270788943703));
#88543=CARTESIAN_POINT('Ctrl Pts',(16.6302310218749,-18.7156480721986,-1.52317526420203));
#88544=CARTESIAN_POINT('Ctrl Pts',(16.6306973521562,-18.7115335408175,-1.52342700864471));
#88545=CARTESIAN_POINT('Ctrl Pts',(16.6320285811685,-18.700088018914,-1.52412938350687));
#88546=CARTESIAN_POINT('Ctrl Pts',(16.6329197472915,-18.6927602272319,-1.52458145350547));
#88547=CARTESIAN_POINT('Ctrl Pts',(16.6382144774426,-18.651044958285,-1.5271680003287));
#88548=CARTESIAN_POINT('Ctrl Pts',(16.6434236342425,-18.6167671986935,-1.52934380418233));
#88549=CARTESIAN_POINT('Ctrl Pts',(16.6625928143832,-18.508584992473,-1.53633889899296));
#88550=CARTESIAN_POINT('Ctrl Pts',(16.6796496639882,-18.4352914324905,-1.54126751716177));
#88551=CARTESIAN_POINT('Ctrl Pts',(16.7543348565868,-18.177423254658,-1.55897625627325));
#88552=CARTESIAN_POINT('Ctrl Pts',(16.8332855111721,-17.9999711949643,-1.5717449037263));
#88553=CARTESIAN_POINT('Ctrl Pts',(16.9464403168688,-17.8176410045259,-1.58492998889398));
#88554=CARTESIAN_POINT('Ctrl Pts',(16.9579092324591,-17.7997666953292,-1.58622484210071));
#88555=CARTESIAN_POINT('Ctrl Pts',(16.974242179433,-17.7751352678872,-1.58801296802193));
#88556=CARTESIAN_POINT('Ctrl Pts',(16.9788797337915,-17.76823015794,-1.58851466901488));
#88557=CARTESIAN_POINT('Ctrl Pts',(16.9869555328482,-17.7563574430456,-1.58937808933288));
#88558=CARTESIAN_POINT('Ctrl Pts',(16.9903745411024,-17.7513769307287,-1.58974053015028));
#88559=CARTESIAN_POINT('Ctrl Pts',(16.9974994157034,-17.7410926615325,-1.59048946944054));
#88560=CARTESIAN_POINT('Ctrl Pts',(17.0012083753689,-17.735791116354,-1.59087584489431));
#88561=CARTESIAN_POINT('Ctrl Pts',(17.009952791334,-17.7234131486053,-1.59177869310054));
#88562=CARTESIAN_POINT('Ctrl Pts',(17.0150076288238,-17.7163505107052,-1.5922944158827));
#88563=CARTESIAN_POINT('Ctrl Pts',(17.031567848859,-17.6935108063976,-1.59396424933792));
#88564=CARTESIAN_POINT('Ctrl Pts',(17.0432482893916,-17.6778614790923,-1.59511157949382));
#88565=CARTESIAN_POINT('Ctrl Pts',(17.1041455636488,-17.5985843175102,-1.60094402637634));
#88566=CARTESIAN_POINT('Ctrl Pts',(17.1567461429151,-17.5376337818345,-1.60549251926172));
#88567=CARTESIAN_POINT('Ctrl Pts',(17.329516956635,-17.3590976113531,-1.61926736492122));
#88568=CARTESIAN_POINT('Ctrl Pts',(17.4602834509425,-17.2527209135448,-1.62810923135766));
#88569=CARTESIAN_POINT('Ctrl Pts',(17.6034467604446,-17.1621563124989,-1.6376217276704));
#88570=CARTESIAN_POINT('Ctrl Pts',(17.6046584667641,-17.1613915127949,-1.6377022319051));
#88571=CARTESIAN_POINT('Ctrl Pts',(17.6514445974002,-17.1319276205065,-1.64081038340964));
#88572=CARTESIAN_POINT('Ctrl Pts',(17.6980928740948,-17.1049794135023,-1.64389968791362));
#88573=CARTESIAN_POINT('Ctrl Pts',(17.7534415275718,-17.0757616215067,-1.64761365576674));
#88574=CARTESIAN_POINT('Ctrl Pts',(17.7611948902049,-17.0717299174897,-1.64813499645596));
#88575=CARTESIAN_POINT('Ctrl Pts',(17.7729668113755,-17.0657008863011,-1.64892851218767));
#88576=CARTESIAN_POINT('Ctrl Pts',(17.7769672333537,-17.0636680856661,-1.64919851184222));
#88577=CARTESIAN_POINT('Ctrl Pts',(17.7841567259295,-17.0600434839143,-1.64968441595113));
#88578=CARTESIAN_POINT('Ctrl Pts',(17.7873433781023,-17.0584470052359,-1.64990002294738));
#88579=CARTESIAN_POINT('Ctrl Pts',(17.7942731678303,-17.0549971200321,-1.65036941252753));
#88580=CARTESIAN_POINT('Ctrl Pts',(17.7980177138375,-17.0531467658083,-1.65062337523431));
#88581=CARTESIAN_POINT('Ctrl Pts',(17.8085431263604,-17.0479843684589,-1.65133809092136));
#88582=CARTESIAN_POINT('Ctrl Pts',(17.8153361833368,-17.0446975231667,-1.65180036515255));
#88583=CARTESIAN_POINT('Ctrl Pts',(17.8558860173623,-17.025344221543,-1.65456511199464));
#88584=CARTESIAN_POINT('Ctrl Pts',(17.8900437993385,-17.0101389880646,-1.65691571542617));
#88585=CARTESIAN_POINT('Ctrl Pts',(18.0033901188386,-16.9632385817009,-1.66474444330013));
#88586=CARTESIAN_POINT('Ctrl Pts',(18.0840901881355,-16.935424153876,-1.67036035145717));
#88587=CARTESIAN_POINT('Ctrl Pts',(18.3376426344206,-16.8648380641333,-1.6877475323215));
#88588=CARTESIAN_POINT('Ctrl Pts',(18.5144120315916,-16.8389099282527,-1.69943894507714));
#88589=CARTESIAN_POINT('Ctrl Pts',(18.7151607496233,-16.8349610471212,-1.71179547501948));
#88590=CARTESIAN_POINT('Ctrl Pts',(18.7379628773226,-16.834880918614,-1.71318717317304));
#88591=CARTESIAN_POINT('Ctrl Pts',(18.7702765490289,-16.8352894524244,-1.71514332247176));
#88592=CARTESIAN_POINT('Ctrl Pts',(18.7797897258551,-16.8354738754609,-1.71571724340865));
#88593=CARTESIAN_POINT('Ctrl Pts',(18.7952605429755,-16.8358781507666,-1.71664745859521));
#88594=CARTESIAN_POINT('Ctrl Pts',(18.8012189891902,-16.8360590406275,-1.71700496868391));
#88595=CARTESIAN_POINT('Ctrl Pts',(18.8137022580778,-16.8364907977761,-1.71775242172126));
#88596=CARTESIAN_POINT('Ctrl Pts',(18.820226852909,-16.8367466898862,-1.71814220320791));
#88597=CARTESIAN_POINT('Ctrl Pts',(18.8357687662672,-16.8374282682119,-1.71906861637003));
#88598=CARTESIAN_POINT('Ctrl Pts',(18.8447847983785,-16.8378814548477,-1.71960438069374));
#88599=CARTESIAN_POINT('Ctrl Pts',(18.8752582740957,-16.8396086695274,-1.72140982073752));
#88600=CARTESIAN_POINT('Ctrl Pts',(18.8966995662194,-16.8411518448067,-1.72267106170812));
#88601=CARTESIAN_POINT('Ctrl Pts',(19.0969103816754,-16.8586302869528,-1.73437240113143));
#88602=CARTESIAN_POINT('Ctrl Pts',(19.2729932943878,-16.89691024181,-1.74401549097663));
#88603=CARTESIAN_POINT('Ctrl Pts',(19.555680165295,-16.9972509061845,-1.76034065820621));
#88604=CARTESIAN_POINT('Ctrl Pts',(19.665548618835,-17.0471611578171,-1.7669501206697));
#88605=CARTESIAN_POINT('Ctrl Pts',(19.7788406048874,-17.1107810285964,-1.77465075512426));
#88606=CARTESIAN_POINT('Ctrl Pts',(19.7870896100963,-17.1154866034291,-1.77521683153408));
#88607=CARTESIAN_POINT('Ctrl Pts',(19.7992701083452,-17.1225439113445,-1.77606112593602));
#88608=CARTESIAN_POINT('Ctrl Pts',(19.8032262087672,-17.1248532358804,-1.776336671653));
#88609=CARTESIAN_POINT('Ctrl Pts',(19.8102536264388,-17.1289860423741,-1.77682856121645));
#88610=CARTESIAN_POINT('Ctrl Pts',(19.813327854645,-17.1308044750554,-1.77704457608362));
#88611=CARTESIAN_POINT('Ctrl Pts',(19.8199297925728,-17.1347321664726,-1.77751027796089));
#88612=CARTESIAN_POINT('Ctrl Pts',(19.8234559143078,-17.1368438901057,-1.77776012057472));
#88613=CARTESIAN_POINT('Ctrl Pts',(19.8331776616163,-17.1427045821478,-1.77845197327704));
#88614=CARTESIAN_POINT('Ctrl Pts',(19.8393601668363,-17.1464750516987,-1.77889535492862));
#88615=CARTESIAN_POINT('Ctrl Pts',(19.8732150762711,-17.1673609015836,-1.78134148895371));
#88616=CARTESIAN_POINT('Ctrl Pts',(19.9005077969649,-17.1850798003169,-1.78338058488923));
#88617=CARTESIAN_POINT('Ctrl Pts',(20.0617667978381,-17.2951366058749,-1.79578659081906));
#88618=CARTESIAN_POINT('Ctrl Pts',(20.1851293400508,-17.4020372440554,-1.80674338849313));
#88619=CARTESIAN_POINT('Ctrl Pts',(20.3739339838297,-17.6081435535026,-1.82500093318393));
#88620=CARTESIAN_POINT('Ctrl Pts',(20.4455825376158,-17.7006700503044,-1.8324416789022));
#88621=CARTESIAN_POINT('Ctrl Pts',(20.5170242133553,-17.8106333459433,-1.84044864655322));
#88622=CARTESIAN_POINT('Ctrl Pts',(20.5246877072974,-17.8226945784887,-1.8413166204403));
#88623=CARTESIAN_POINT('Ctrl Pts',(20.5366901870894,-17.8420141587161,-1.84269092574387));
#88624=CARTESIAN_POINT('Ctrl Pts',(20.5411087188692,-17.8492223433959,-1.84320018521964));
#88625=CARTESIAN_POINT('Ctrl Pts',(20.5488253331642,-17.8619817895322,-1.84409556143304));
#88626=CARTESIAN_POINT('Ctrl Pts',(20.552141399816,-17.8675219961872,-1.84448233429578));
#88627=CARTESIAN_POINT('Ctrl Pts',(20.5589476646209,-17.8790122999689,-1.8452804014591));
#88628=CARTESIAN_POINT('Ctrl Pts',(20.5624342350925,-17.88496446512,-1.84569156037906));
#88629=CARTESIAN_POINT('Ctrl Pts',(20.5713091019736,-17.9002865930589,-1.84674426816887));
#88630=CARTESIAN_POINT('Ctrl Pts',(20.5766548865702,-17.9096810458922,-1.84738427573947));
#88631=CARTESIAN_POINT('Ctrl Pts',(20.5986660020505,-17.9490610492703,-1.85004493600299));
#88632=CARTESIAN_POINT('Ctrl Pts',(20.6146737458542,-17.9794094919502,-1.85204205999933));
#88633=CARTESIAN_POINT('Ctrl Pts',(20.6544540153659,-18.059485616522,-1.85718612639655));
#88634=CARTESIAN_POINT('Ctrl Pts',(20.6770353996593,-18.1097769708,-1.86029367990828));
#88635=CARTESIAN_POINT('Ctrl Pts',(20.7384916002391,-18.2623196121299,-1.86943807922409));
#88636=CARTESIAN_POINT('Ctrl Pts',(20.7714349183699,-18.3667603483404,-1.8753261953939));
#88637=CARTESIAN_POINT('Ctrl Pts',(20.8065014060671,-18.5178142363522,-1.88376889397428));
#88638=CARTESIAN_POINT('Ctrl Pts',(20.8153945084739,-18.5626723507075,-1.88626879020511));
#88639=CARTESIAN_POINT('Ctrl Pts',(20.8265372287805,-18.6302900001255,-1.89006877648479));
#88640=CARTESIAN_POINT('Ctrl Pts',(20.8298822214581,-18.6528561555841,-1.89134223616384));
#88641=CARTESIAN_POINT('Ctrl Pts',(20.8330041677115,-18.6765518350039,-1.89268888892799));
#88642=CARTESIAN_POINT('Ctrl Pts',(20.8331456863524,-18.677632408744,-1.89275031974608));
#88643=CARTESIAN_POINT('Ctrl Pts',(20.8357822149616,-18.6978852213276,-1.89390208910439));
#88644=CARTESIAN_POINT('Ctrl Pts',(20.8380152338742,-18.7170901156452,-1.89500086273349));
#88645=CARTESIAN_POINT('Ctrl Pts',(20.8433022300961,-18.7687150004179,-1.89797846519824));
#88646=CARTESIAN_POINT('Ctrl Pts',(20.8458716164511,-18.8011779070191,-1.89987614786798));
#88647=CARTESIAN_POINT('Ctrl Pts',(20.84807483845,-18.8405383825168,-1.90222141491291));
#88648=CARTESIAN_POINT('Ctrl Pts',(20.8484251155452,-18.8473933913309,-1.90263149309796));
#88649=CARTESIAN_POINT('Ctrl Pts',(20.8489464635304,-18.8586723182389,-1.90330907026286));
#88650=CARTESIAN_POINT('Ctrl Pts',(20.849137007669,-18.8630953445978,-1.90357550317239));
#88651=CARTESIAN_POINT('Ctrl Pts',(20.8494557736874,-18.8710768935609,-1.90405764659642));
#88652=CARTESIAN_POINT('Ctrl Pts',(20.8495888923784,-18.8746351650505,-1.90427308002196));
#88653=CARTESIAN_POINT('Ctrl Pts',(20.8498603283221,-18.8824160900512,-1.90474524763149));
#88654=CARTESIAN_POINT('Ctrl Pts',(20.8499949809104,-18.8866387765287,-1.90500217933183));
#88655=CARTESIAN_POINT('Ctrl Pts',(20.8503413494707,-18.8986272932997,-1.90573352465153));
#88656=CARTESIAN_POINT('Ctrl Pts',(20.850522956719,-18.9063938305408,-1.90620957280006));
#88657=CARTESIAN_POINT('Ctrl Pts',(20.8514032121794,-18.9556341826149,-1.90924132112767));
#88658=CARTESIAN_POINT('Ctrl Pts',(20.8509254808769,-18.9971170656735,-1.91185635046042));
#88659=CARTESIAN_POINT('Ctrl Pts',(20.8415154411867,-19.2270774408199,-1.9265951086465));
#88660=CARTESIAN_POINT('Ctrl Pts',(20.8086346485021,-19.4137259082036,-1.93936820897715));
#88661=CARTESIAN_POINT('Ctrl Pts',(20.742225650577,-19.6225553661527,-1.95345843539751));
#88662=CARTESIAN_POINT('Ctrl Pts',(20.7323805677967,-19.6513496975902,-1.9553992464878));
#88663=CARTESIAN_POINT('Ctrl Pts',(20.7030258713015,-19.7315157831484,-1.960794254304));
#88664=CARTESIAN_POINT('Ctrl Pts',(20.6821313652457,-19.7823570290993,-1.96420534021535));
#88665=CARTESIAN_POINT('Ctrl Pts',(20.6543086333005,-19.8432052003897,-1.96827775162737));
#88666=CARTESIAN_POINT('Ctrl Pts',(20.6492445721393,-19.8540366923927,-1.96900231598644));
#88667=CARTESIAN_POINT('Ctrl Pts',(20.6407076163965,-19.8719002992084,-1.97019683697838));
#88668=CARTESIAN_POINT('Ctrl Pts',(20.6372869747759,-19.8789569510705,-1.97066859078805));
#88669=CARTESIAN_POINT('Ctrl Pts',(20.6310186624264,-19.8917072509704,-1.97152082030682));
#88670=CARTESIAN_POINT('Ctrl Pts',(20.6281843830802,-19.897407344686,-1.97190175676418));
#88671=CARTESIAN_POINT('Ctrl Pts',(20.6220398102003,-19.909626297976,-1.97271826294207));
#88672=CARTESIAN_POINT('Ctrl Pts',(20.6187213637344,-19.9161409827491,-1.97315354101601));
#88673=CARTESIAN_POINT('Ctrl Pts',(20.6095568407958,-19.9339043960364,-1.97434034252751));
#88674=CARTESIAN_POINT('Ctrl Pts',(20.6036433092963,-19.9451181261748,-1.97508948241279));
#88675=CARTESIAN_POINT('Ctrl Pts',(20.5714518772119,-20.0048554513749,-1.97908088540586));
#88676=CARTESIAN_POINT('Ctrl Pts',(20.543383744079,-20.0523932187758,-1.98225856180017));
#88677=CARTESIAN_POINT('Ctrl Pts',(20.4045754762848,-20.2677850080817,-1.99676178879126));
#88678=CARTESIAN_POINT('Ctrl Pts',(20.2721580848393,-20.4203910497828,-2.00723938597097));
#88679=CARTESIAN_POINT('Ctrl Pts',(20.0760807655472,-20.5902669747901,-2.02177024819191));
#88680=CARTESIAN_POINT('Ctrl Pts',(20.0303833966853,-20.6266606372342,-2.02510930740973));
#88681=CARTESIAN_POINT('Ctrl Pts',(19.9760513928753,-20.6663735688224,-2.02910148379458));
#88682=CARTESIAN_POINT('Ctrl Pts',(19.9688247502487,-20.6715860623682,-2.0296329185514));
#88683=CARTESIAN_POINT('Ctrl Pts',(19.9578797944069,-20.679375962364,-2.03043880605199));
#88684=CARTESIAN_POINT('Ctrl Pts',(19.954185667365,-20.6819873996058,-2.03071098081464));
#88685=CARTESIAN_POINT('Ctrl Pts',(19.9475640087384,-20.686636595846,-2.03119921254773));
#88686=CARTESIAN_POINT('Ctrl Pts',(19.9446396727346,-20.6886788147173,-2.03141495967418));
#88687=CARTESIAN_POINT('Ctrl Pts',(19.9383021034834,-20.6930808890209,-2.03188281384409));
#88688=CARTESIAN_POINT('Ctrl Pts',(19.9348871363444,-20.6954380699205,-2.03213509104795));
#88689=CARTESIAN_POINT('Ctrl Pts',(19.92534527731,-20.70198300181,-2.03284042616234));
#88690=CARTESIAN_POINT('Ctrl Pts',(19.9192033315884,-20.7061485499906,-2.03329494306932));
#88691=CARTESIAN_POINT('Ctrl Pts',(19.883722832002,-20.7299404824401,-2.03592286957803));
#88692=CARTESIAN_POINT('Ctrl Pts',(19.8539207880316,-20.7488617197514,-2.03813913853463));
#88693=CARTESIAN_POINT('Ctrl Pts',(19.7572519413887,-20.8068973882745,-2.04532195273009));
#88694=CARTESIAN_POINT('Ctrl Pts',(19.6887082243677,-20.8430894835651,-2.05040399350328));
#88695=CARTESIAN_POINT('Ctrl Pts',(19.4459888701783,-20.9546845728264,-2.06803347255593));
#88696=CARTESIAN_POINT('Ctrl Pts',(19.2637255529462,-21.0104202644713,-2.08055055417731));
#88697=CARTESIAN_POINT('Ctrl Pts',(19.0550779585259,-21.0446220455466,-2.09354732554634));
#88698=CARTESIAN_POINT('Ctrl Pts',(19.0336518283081,-21.0477974418953,-2.09486833251379));
#88699=CARTESIAN_POINT('Ctrl Pts',(19.0038655028294,-21.0517456887764,-2.09668649192162));
#88700=CARTESIAN_POINT('Ctrl Pts',(18.9955443399767,-21.0527983978826,-2.09719244640404));
#88701=CARTESIAN_POINT('Ctrl Pts',(18.9812014007374,-21.0545263805028,-2.09806121414425));
#88702=CARTESIAN_POINT('Ctrl Pts',(18.9751826239734,-21.0552252985158,-2.09842476978755));
#88703=CARTESIAN_POINT('Ctrl Pts',(18.9627416061524,-21.0566158793265,-2.09917420018124));
#88704=CARTESIAN_POINT('Ctrl Pts',(18.956319027622,-21.0573040097057,-2.09955995987141));
#88705=CARTESIAN_POINT('Ctrl Pts',(18.941319896432,-21.0588416497312,-2.10045826831727));
#88706=CARTESIAN_POINT('Ctrl Pts',(18.9327410661623,-21.0596682064475,-2.1009700895789));
#88707=CARTESIAN_POINT('Ctrl Pts',(18.9050768148987,-21.0621632047661,-2.10261438659748));
#88708=CARTESIAN_POINT('Ctrl Pts',(18.8859733772833,-21.0636250035493,-2.10374037181206));
#88709=CARTESIAN_POINT('Ctrl Pts',(18.7060367786558,-21.0749392184033,-2.11426346527496));
#88710=CARTESIAN_POINT('Ctrl Pts',(18.5445898530113,-21.0666594822605,-2.12302931712828));
#88711=CARTESIAN_POINT('Ctrl Pts',(18.3790956223689,-21.0390495329574,-2.13214074052811));
#88712=CARTESIAN_POINT('Ctrl Pts',(18.3725676077833,-21.0379289288149,-2.13250044424435));
#88713=CARTESIAN_POINT('Ctrl Pts',(18.3040941985539,-21.0258436423303,-2.13627738645831));
#88714=CARTESIAN_POINT('Ctrl Pts',(18.2426636085114,-21.012153992812,-2.13969897445675));
#88715=CARTESIAN_POINT('Ctrl Pts',(18.16033766413,-20.9899158601766,-2.1444281328191));
#88716=CARTESIAN_POINT('Ctrl Pts',(18.1388336305284,-20.9837397649306,-2.14567707794279));
#88717=CARTESIAN_POINT('Ctrl Pts',(18.068302377477,-20.9622669278466,-2.14983037512416));
#88718=CARTESIAN_POINT('Ctrl Pts',(18.019737415036,-20.9455281503479,-2.15278144658085));
#88719=CARTESIAN_POINT('Ctrl Pts',(17.9644860062333,-20.9242066923814,-2.15629650326148));
#88720=CARTESIAN_POINT('Ctrl Pts',(17.9571545816596,-20.9213303978051,-2.15676618659363));
#88721=CARTESIAN_POINT('Ctrl Pts',(17.9454906688202,-20.9166790970874,-2.15751890115621));
#88722=CARTESIAN_POINT('Ctrl Pts',(17.9411476445557,-20.9149304779826,-2.15780038808813));
#88723=CARTESIAN_POINT('Ctrl Pts',(17.9334819694323,-20.9118144791046,-2.15829943990884));
#88724=CARTESIAN_POINT('Ctrl Pts',(17.9301569547186,-20.9104530293502,-2.15851664503251));
#88725=CARTESIAN_POINT('Ctrl Pts',(17.9231343395083,-20.9075566747733,-2.15897698170939));
#88726=CARTESIAN_POINT('Ctrl Pts',(17.9194376800836,-20.9060197680609,-2.15922022824439));
#88727=CARTESIAN_POINT('Ctrl Pts',(17.9096363108687,-20.9019121478584,-2.15986759874973));
#88728=CARTESIAN_POINT('Ctrl Pts',(17.903539326646,-20.8993232766162,-2.16027280075813));
#88729=CARTESIAN_POINT('Ctrl Pts',(17.8745153525016,-20.8868381651829,-2.16221332577391));
#88730=CARTESIAN_POINT('Ctrl Pts',(17.8517535552687,-20.8765658389402,-2.16376981215767));
#88731=CARTESIAN_POINT('Ctrl Pts',(17.7878648028456,-20.8463615398583,-2.16822656341672));
#88732=CARTESIAN_POINT('Ctrl Pts',(17.7471954762113,-20.8254977315505,-2.17116834600413));
#88733=CARTESIAN_POINT('Ctrl Pts',(17.6162479728418,-20.7528733084796,-2.18091824183866));
#88734=CARTESIAN_POINT('Ctrl Pts',(17.5291052774362,-20.6957725579613,-2.1878464578787));
#88735=CARTESIAN_POINT('Ctrl Pts',(17.4082739301036,-20.6031995852273,-2.19785403650203));
#88736=CARTESIAN_POINT('Ctrl Pts',(17.3710430952452,-20.572604367932,-2.20100111399996));
#88737=CARTESIAN_POINT('Ctrl Pts',(17.2665817762122,-20.4806126403095,-2.20999133998629));
#88738=CARTESIAN_POINT('Ctrl Pts',(17.2022198594721,-20.4161127904904,-2.21572963037585));
#88739=CARTESIAN_POINT('Ctrl Pts',(17.1331431674519,-20.3373285685086,-2.22212281904182));
#88740=CARTESIAN_POINT('Ctrl Pts',(17.1241842624665,-20.3269076864318,-2.2229571073976));
#88741=CARTESIAN_POINT('Ctrl Pts',(17.1099813555459,-20.3100578946565,-2.22428825044668));
#88742=CARTESIAN_POINT('Ctrl Pts',(17.1046726808629,-20.3036842430632,-2.22478775387328));
#88743=CARTESIAN_POINT('Ctrl Pts',(17.0953144889517,-20.2923134563686,-2.22567184531886));
#88744=CARTESIAN_POINT('Ctrl Pts',(17.0912500513045,-20.2873287883209,-2.22605703735929));
#88745=CARTESIAN_POINT('Ctrl Pts',(17.0828301025854,-20.2769058506258,-2.22685758995079));
#88746=CARTESIAN_POINT('Ctrl Pts',(17.0784785900895,-20.2714644391807,-2.22727278660493));
#88747=CARTESIAN_POINT('Ctrl Pts',(17.0672500840754,-20.2572805971603,-2.22834803722952));
#88748=CARTESIAN_POINT('Ctrl Pts',(17.0604149301437,-20.2485052027094,-2.22900641839605));
#88749=CARTESIAN_POINT('Ctrl Pts',(17.0310548901661,-20.2101918694923,-2.23185181854944));
#88750=CARTESIAN_POINT('Ctrl Pts',(17.0092396348382,-20.1801167525585,-2.23401093391364));
#88751=CARTESIAN_POINT('Ctrl Pts',(16.9324166012404,-20.0681186760313,-2.24180569687976));
#88752=CARTESIAN_POINT('Ctrl Pts',(16.8823605285191,-19.9829498781371,-2.24726112357411));
#88753=CARTESIAN_POINT('Ctrl Pts',(16.8038714931498,-19.8251066139317,-2.2568815426041));
#88754=CARTESIAN_POINT('Ctrl Pts',(16.7731660847066,-19.7537739034998,-2.26106805065016));
#88755=CARTESIAN_POINT('Ctrl Pts',(16.746103513988,-19.6799818359296,-2.26536490179543));
#88756=CARTESIAN_POINT('Ctrl Pts',(16.7457611493293,-19.679046260681,-2.26541937453551));
#88757=CARTESIAN_POINT('Ctrl Pts',(16.7454194499845,-19.6781104572309,-2.26547385582022));
#88758=CARTESIAN_POINT('Ctrl Pts',(16.7454194493934,-19.6781104556121,-2.04625066941376));
#88759=CARTESIAN_POINT('Ctrl Pts',(16.7489322042769,-19.6877307495858,-2.04566730752196));
#88760=CARTESIAN_POINT('Ctrl Pts',(16.7525149176216,-19.6973259561389,-2.04508119867915));
#88761=CARTESIAN_POINT('Ctrl Pts',(16.7671937064808,-19.7357845184218,-2.04271339922677));
#88762=CARTESIAN_POINT('Ctrl Pts',(16.7788510681905,-19.7644269782853,-2.04090763254374));
#88763=CARTESIAN_POINT('Ctrl Pts',(16.7939618142905,-19.799343877772,-2.03864174812154));
#88764=CARTESIAN_POINT('Ctrl Pts',(16.7968258180322,-19.8058711815232,-2.03821535303688));
#88765=CARTESIAN_POINT('Ctrl Pts',(16.8013829451204,-19.8161163158947,-2.03754146458505));
#88766=CARTESIAN_POINT('Ctrl Pts',(16.8030539897001,-19.8198439910864,-2.0372953031527));
#88767=CARTESIAN_POINT('Ctrl Pts',(16.8062079246767,-19.8268254112815,-2.03683241629392));
#88768=CARTESIAN_POINT('Ctrl Pts',(16.8076882727646,-19.8300802439065,-2.03661584705281));
#88769=CARTESIAN_POINT('Ctrl Pts',(16.8111000197593,-19.83753148228,-2.03611831334066));
#88770=CARTESIAN_POINT('Ctrl Pts',(16.8130369074569,-19.8417253150674,-2.03583701398533));
#88771=CARTESIAN_POINT('Ctrl Pts',(16.8190812869548,-19.8547011230306,-2.0349628074716));
#88772=CARTESIAN_POINT('Ctrl Pts',(16.823235323712,-19.8634611010553,-2.03436713444438));
#88773=CARTESIAN_POINT('Ctrl Pts',(16.8705007704965,-19.9613906274576,-2.02764872667878));
#88774=CARTESIAN_POINT('Ctrl Pts',(16.9197541448603,-20.0474479169737,-2.02119664022092));
#88775=CARTESIAN_POINT('Ctrl Pts',(17.0685229099909,-20.2696614655017,-2.00358061007281));
#88776=CARTESIAN_POINT('Ctrl Pts',(17.1785833180263,-20.3979396429235,-1.99239379543893));
#88777=CARTESIAN_POINT('Ctrl Pts',(17.3255701391486,-20.5328156825826,-1.97986693659284));
#88778=CARTESIAN_POINT('Ctrl Pts',(17.3489054613338,-20.5533013993503,-1.97793721896634));
#88779=CARTESIAN_POINT('Ctrl Pts',(17.3842828575061,-20.5830064443116,-1.97509725632832));
#88780=CARTESIAN_POINT('Ctrl Pts',(17.395986180175,-20.5926210478915,-1.97417117321999));
#88781=CARTESIAN_POINT('Ctrl Pts',(17.4148934815203,-20.6078170193875,-1.97269612455211));
#88782=CARTESIAN_POINT('Ctrl Pts',(17.422031901074,-20.6134787751463,-1.97214394376681));
#88783=CARTESIAN_POINT('Ctrl Pts',(17.4357160690194,-20.6241890329257,-1.97109431184133));
#88784=CARTESIAN_POINT('Ctrl Pts',(17.442255254385,-20.6292456118536,-1.97059654411106));
#88785=CARTESIAN_POINT('Ctrl Pts',(17.4537843402227,-20.6380533295884,-1.96972554579386));
#88786=CARTESIAN_POINT('Ctrl Pts',(17.4587614956294,-20.6418209147777,-1.96935166816042));
#88787=CARTESIAN_POINT('Ctrl Pts',(17.4686168009528,-20.6492128003572,-1.96861551823935));
#88788=CARTESIAN_POINT('Ctrl Pts',(17.4734940342832,-20.6528382173812,-1.96825320437367));
#88789=CARTESIAN_POINT('Ctrl Pts',(17.4851944062822,-20.6614575401038,-1.96738873621035));
#88790=CARTESIAN_POINT('Ctrl Pts',(17.4920320191164,-20.6664316929905,-1.96688735184414));
#88791=CARTESIAN_POINT('Ctrl Pts',(17.5168351183849,-20.6842489267646,-1.96508210256015));
#88792=CARTESIAN_POINT('Ctrl Pts',(17.5349718879817,-20.6968519518936,-1.96378745037299));
#88793=CARTESIAN_POINT('Ctrl Pts',(17.7074882102058,-20.8127710615573,-1.95169893375997));
#88794=CARTESIAN_POINT('Ctrl Pts',(17.8746326967339,-20.8956278545903,-1.94176357574396));
#88795=CARTESIAN_POINT('Ctrl Pts',(18.126205239552,-20.9814531380444,-1.92727266167189));
#88796=CARTESIAN_POINT('Ctrl Pts',(18.2033517901554,-21.0029765934799,-1.92287097926848));
#88797=CARTESIAN_POINT('Ctrl Pts',(18.3166937727788,-21.0277746973354,-1.9162341472376));
#88798=CARTESIAN_POINT('Ctrl Pts',(18.3520512099398,-21.0345704922844,-1.91414004919831));
#88799=CARTESIAN_POINT('Ctrl Pts',(18.3949261222642,-21.0416826611219,-1.91155364284013));
#88800=CARTESIAN_POINT('Ctrl Pts',(18.4022962792941,-21.0428652172394,-1.91110737185292));
#88801=CARTESIAN_POINT('Ctrl Pts',(18.4137822629527,-21.0446459083493,-1.91040906938291));
#88802=CARTESIAN_POINT('Ctrl Pts',(18.4178939427768,-21.0452709468089,-1.91015853496584));
#88803=CARTESIAN_POINT('Ctrl Pts',(18.4255344371366,-21.0464093947285,-1.9096918964591));
#88804=CARTESIAN_POINT('Ctrl Pts',(18.4290627166577,-21.0469260055718,-1.90947597580671));
#88805=CARTESIAN_POINT('Ctrl Pts',(18.4370574613303,-21.0480759716808,-1.90898574519351));
#88806=CARTESIAN_POINT('Ctrl Pts',(18.4415246333013,-21.0487039632081,-1.90871113750847));
#88807=CARTESIAN_POINT('Ctrl Pts',(18.4530651639789,-21.0502887232309,-1.9080000067286));
#88808=CARTESIAN_POINT('Ctrl Pts',(18.4601413492167,-21.0512239957201,-1.9075623160122));
#88809=CARTESIAN_POINT('Ctrl Pts',(18.503651929787,-21.0567511303766,-1.90486141668591));
#88810=CARTESIAN_POINT('Ctrl Pts',(18.5401936350737,-21.0604298119851,-1.90255187832858));
#88811=CARTESIAN_POINT('Ctrl Pts',(18.7466642944294,-21.0758029792542,-1.88933830343072));
#88812=CARTESIAN_POINT('Ctrl Pts',(18.9174225550322,-21.0679061203798,-1.87784605114837));
#88813=CARTESIAN_POINT('Ctrl Pts',(19.1795609411833,-21.023782620099,-1.86057005990105));
#88814=CARTESIAN_POINT('Ctrl Pts',(19.2725577202418,-21.0015774257592,-1.85450266049592));
#88815=CARTESIAN_POINT('Ctrl Pts',(19.3841839191674,-20.9667972656394,-1.84732074826407));
#88816=CARTESIAN_POINT('Ctrl Pts',(19.4045222174015,-20.9601203049497,-1.8460160539593));
#88817=CARTESIAN_POINT('Ctrl Pts',(19.4332751455721,-20.9501953075874,-1.84417646704904));
#88818=CARTESIAN_POINT('Ctrl Pts',(19.4417751705084,-20.9472003729995,-1.84363325479264));
#88819=CARTESIAN_POINT('Ctrl Pts',(19.4563977975804,-20.9419429693114,-1.84269974633085));
#88820=CARTESIAN_POINT('Ctrl Pts',(19.4625294869523,-20.9397063131113,-1.84230859846981));
#88821=CARTESIAN_POINT('Ctrl Pts',(19.4742444575106,-20.9353715527305,-1.84156182341194));
#88822=CARTESIAN_POINT('Ctrl Pts',(19.4798293983894,-20.9332781436928,-1.84120604402413));
#88823=CARTESIAN_POINT('Ctrl Pts',(19.4943170105604,-20.9277777977739,-1.84028370387048));
#88824=CARTESIAN_POINT('Ctrl Pts',(19.503205714463,-20.9243342607374,-1.83971837377366));
#88825=CARTESIAN_POINT('Ctrl Pts',(19.5333737536923,-20.9124120193906,-1.83780132305922));
#88826=CARTESIAN_POINT('Ctrl Pts',(19.5545390778004,-20.9036478590996,-1.83645921105149));
#88827=CARTESIAN_POINT('Ctrl Pts',(19.7376084146322,-20.8243375502823,-1.82486496401925));
#88828=CARTESIAN_POINT('Ctrl Pts',(19.8902352961146,-20.7341347697657,-1.8153749742479));
#88829=CARTESIAN_POINT('Ctrl Pts',(20.0980782170554,-20.5732382974583,-1.80107084229505));
#88830=CARTESIAN_POINT('Ctrl Pts',(20.1629639637541,-20.5163473527647,-1.79634826998978));
#88831=CARTESIAN_POINT('Ctrl Pts',(20.2509188782263,-20.4291803186487,-1.78927674433768));
#88832=CARTESIAN_POINT('Ctrl Pts',(20.2769299780823,-20.4019900917892,-1.78709093369609));
#88833=CARTESIAN_POINT('Ctrl Pts',(20.3072797516479,-20.3685228489651,-1.78440282271994));
#88834=CARTESIAN_POINT('Ctrl Pts',(20.3123283810147,-20.3628953456445,-1.78395089266901));
#88835=CARTESIAN_POINT('Ctrl Pts',(20.3201211831639,-20.3541148537573,-1.78324564659932));
#88836=CARTESIAN_POINT('Ctrl Pts',(20.3228864021304,-20.3509805113868,-1.78299387619146));
#88837=CARTESIAN_POINT('Ctrl Pts',(20.327992186836,-20.345158501459,-1.78252613113828));
#88838=CARTESIAN_POINT('Ctrl Pts',(20.3303352547559,-20.3424731049976,-1.78231034749362));
#88839=CARTESIAN_POINT('Ctrl Pts',(20.3356104994543,-20.3363962249681,-1.78182196459464));
#88840=CARTESIAN_POINT('Ctrl Pts',(20.3385386735938,-20.3330013554498,-1.78154907719995));
#88841=CARTESIAN_POINT('Ctrl Pts',(20.3471307612879,-20.3229756363641,-1.78074310563295));
#88842=CARTESIAN_POINT('Ctrl Pts',(20.3527644316675,-20.3163191552111,-1.78020788444492));
#88843=CARTESIAN_POINT('Ctrl Pts',(20.3925765091302,-20.2686853366594,-1.77637829095071));
#88844=CARTESIAN_POINT('Ctrl Pts',(20.425233109386,-20.2264668866777,-1.77298679910305));
#88845=CARTESIAN_POINT('Ctrl Pts',(20.4665197727916,-20.1687069051944,-1.76839817527937));
#88846=CARTESIAN_POINT('Ctrl Pts',(20.4766022656412,-20.1542220159567,-1.76725152215736));
#88847=CARTESIAN_POINT('Ctrl Pts',(20.5136850673665,-20.0995007462578,-1.76293918727684));
#88848=CARTESIAN_POINT('Ctrl Pts',(20.5394820045799,-20.0584679821908,-1.75974486644343));
#88849=CARTESIAN_POINT('Ctrl Pts',(20.6188535390919,-19.9220415972636,-1.74931868869326));
#88850=CARTESIAN_POINT('Ctrl Pts',(20.6664533299026,-19.8233674069179,-1.74208589179603));
#88851=CARTESIAN_POINT('Ctrl Pts',(20.726242996681,-19.6701176975957,-1.73151223824997));
#88852=CARTESIAN_POINT('Ctrl Pts',(20.7442598175681,-19.61801912314,-1.72802300249035));
#88853=CARTESIAN_POINT('Ctrl Pts',(20.7701617717284,-19.5324403361156,-1.72246530201314));
#88854=CARTESIAN_POINT('Ctrl Pts',(20.7793001312507,-19.4993694674331,-1.72035839536925));
#88855=CARTESIAN_POINT('Ctrl Pts',(20.7902558605439,-19.4556046636963,-1.71762182929286));
#88856=CARTESIAN_POINT('Ctrl Pts',(20.7928002588466,-19.4450997082502,-1.71696882716814));
#88857=CARTESIAN_POINT('Ctrl Pts',(20.796836531,-19.4278592520601,-1.71590333490508));
#88858=CARTESIAN_POINT('Ctrl Pts',(20.798376109843,-19.4211352259861,-1.71548931529222));
#88859=CARTESIAN_POINT('Ctrl Pts',(20.8012930918354,-19.4081030150994,-1.71468981237898));
#88860=CARTESIAN_POINT('Ctrl Pts',(20.8026745525849,-19.4017958257325,-1.71430420272409));
#88861=CARTESIAN_POINT('Ctrl Pts',(20.8057982323911,-19.3872155344339,-1.71341580275816));
#88862=CARTESIAN_POINT('Ctrl Pts',(20.8075197981364,-19.378938083393,-1.71291367847392));
#88863=CARTESIAN_POINT('Ctrl Pts',(20.8120175439487,-19.3566433861434,-1.71156711253913));
#88864=CARTESIAN_POINT('Ctrl Pts',(20.8147014981895,-19.3426078253813,-1.71072561209479));
#88865=CARTESIAN_POINT('Ctrl Pts',(20.8380194335241,-19.2136011640022,-1.70304550942558));
#88866=CARTESIAN_POINT('Ctrl Pts',(20.8492485225456,-19.0971271651064,-1.69652342597104));
#88867=CARTESIAN_POINT('Ctrl Pts',(20.852986022774,-18.8176429758351,-1.68122171400578));
#88868=CARTESIAN_POINT('Ctrl Pts',(20.8364045221451,-18.6552897483496,-1.67262496729782));
#88869=CARTESIAN_POINT('Ctrl Pts',(20.7943954072476,-18.4646383929559,-1.66141638514543));
#88870=CARTESIAN_POINT('Ctrl Pts',(20.7866511669756,-18.4329879635266,-1.65951617515095));
#88871=CARTESIAN_POINT('Ctrl Pts',(20.7762964575871,-18.3945355054772,-1.65714514738014));
#88872=CARTESIAN_POINT('Ctrl Pts',(20.7743768450401,-18.3875499932671,-1.65671186957185));
#88873=CARTESIAN_POINT('Ctrl Pts',(20.7713118682583,-18.3766164326263,-1.65602952505341));
#88874=CARTESIAN_POINT('Ctrl Pts',(20.7701907735971,-18.372661557458,-1.65578184655573));
#88875=CARTESIAN_POINT('Ctrl Pts',(20.7680740731689,-18.3652765369688,-1.65531769667394));
#88876=CARTESIAN_POINT('Ctrl Pts',(20.767081303078,-18.3618456374567,-1.65510139106755));
#88877=CARTESIAN_POINT('Ctrl Pts',(20.7647957461462,-18.3540212281235,-1.65460656268978));
#88878=CARTESIAN_POINT('Ctrl Pts',(20.7634973863276,-18.3496294062956,-1.65432771862164));
#88879=CARTESIAN_POINT('Ctrl Pts',(20.7594644043921,-18.3361485275235,-1.65346849318304));
#88880=CARTESIAN_POINT('Ctrl Pts',(20.7566829421758,-18.3270737664884,-1.65288547812979));
#88881=CARTESIAN_POINT('Ctrl Pts',(20.7312360812672,-18.2460010856649,-1.64763738004858));
#88882=CARTESIAN_POINT('Ctrl Pts',(20.7047984183217,-18.1752519623246,-1.64277935846478));
#88883=CARTESIAN_POINT('Ctrl Pts',(20.6205227880263,-17.9819147909825,-1.62898784800352));
#88884=CARTESIAN_POINT('Ctrl Pts',(20.5546065873095,-17.8632259766173,-1.61993455239341));
#88885=CARTESIAN_POINT('Ctrl Pts',(20.4268036808233,-17.6775610453561,-1.60532712693758));
#88886=CARTESIAN_POINT('Ctrl Pts',(20.3711302633979,-17.6067910745857,-1.59962724702033));
#88887=CARTESIAN_POINT('Ctrl Pts',(20.2972856710032,-17.5243247070143,-1.59283221782233));
#88888=CARTESIAN_POINT('Ctrl Pts',(20.2832287957971,-17.5090831563693,-1.59156906340394));
#88889=CARTESIAN_POINT('Ctrl Pts',(20.2628224658996,-17.4875990887467,-1.58977744674432));
#88890=CARTESIAN_POINT('Ctrl Pts',(20.2566543662652,-17.4811866720112,-1.58924124340499));
#88891=CARTESIAN_POINT('Ctrl Pts',(20.2459061214758,-17.4701527710375,-1.58831598793813));
#88892=CARTESIAN_POINT('Ctrl Pts',(20.241344794358,-17.4655132013609,-1.58792612370734));
#88893=CARTESIAN_POINT('Ctrl Pts',(20.2325437817913,-17.4566433863577,-1.58717919205395));
#88894=CARTESIAN_POINT('Ctrl Pts',(20.2283073981052,-17.4524099663535,-1.58682198496484));
#88895=CARTESIAN_POINT('Ctrl Pts',(20.2171857297862,-17.4413900062779,-1.58589024093901));
#88896=CARTESIAN_POINT('Ctrl Pts',(20.2102717719477,-17.434632502577,-1.58531698576174));
#88897=CARTESIAN_POINT('Ctrl Pts',(20.1862331043846,-17.4114576343401,-1.58334411946047));
#88898=CARTESIAN_POINT('Ctrl Pts',(20.1688785050395,-17.3952805286651,-1.58195490273184));
#88899=CARTESIAN_POINT('Ctrl Pts',(20.0307355927917,-17.2707838304731,-1.57115663692911));
#88900=CARTESIAN_POINT('Ctrl Pts',(19.8981299120915,-17.17638192739,-1.56237387389386));
#88901=CARTESIAN_POINT('Ctrl Pts',(19.6418773318728,-17.0351175034129,-1.54647744047427));
#88902=CARTESIAN_POINT('Ctrl Pts',(19.5221729686457,-16.9828750013885,-1.53938838462176));
#88903=CARTESIAN_POINT('Ctrl Pts',(19.3871558638748,-16.9382428548846,-1.53099654513051));
#88904=CARTESIAN_POINT('Ctrl Pts',(19.3758337329098,-16.9346056739711,-1.53028982396407));
#88905=CARTESIAN_POINT('Ctrl Pts',(19.3596897369035,-16.9295691476304,-1.52927706601121));
#88906=CARTESIAN_POINT('Ctrl Pts',(19.3548923729526,-16.9280911928868,-1.52897548174137));
#88907=CARTESIAN_POINT('Ctrl Pts',(19.3466139669694,-16.9255730145929,-1.52845390213791));
#88908=CARTESIAN_POINT('Ctrl Pts',(19.3431353839694,-16.9245246527862,-1.52823438145548));
#88909=CARTESIAN_POINT('Ctrl Pts',(19.3363837882651,-16.9225088272918,-1.52780760180038));
#88910=CARTESIAN_POINT('Ctrl Pts',(19.333111127962,-16.921540321889,-1.5276004110663));
#88911=CARTESIAN_POINT('Ctrl Pts',(19.324271786898,-16.9189476534943,-1.52703995934316));
#88912=CARTESIAN_POINT('Ctrl Pts',(19.3187007994672,-16.9173384558301,-1.52668584075044));
#88913=CARTESIAN_POINT('Ctrl Pts',(19.2979796407993,-16.9114452110633,-1.52536556985298));
#88914=CARTESIAN_POINT('Ctrl Pts',(19.2827888656673,-16.9073074487301,-1.52439146148075));
#88915=CARTESIAN_POINT('Ctrl Pts',(19.1401771138437,-16.8701655900877,-1.51519762888554));
#88916=CARTESIAN_POINT('Ctrl Pts',(19.0099955933185,-16.8489463441904,-1.50645979768121));
#88917=CARTESIAN_POINT('Ctrl Pts',(18.7197391250688,-16.8290602835138,-1.48724159268695));
#88918=CARTESIAN_POINT('Ctrl Pts',(18.5600276785025,-16.8361483424727,-1.47686847792856));
#88919=CARTESIAN_POINT('Ctrl Pts',(18.3815830380192,-16.8644310420887,-1.46577185052176));
#88920=CARTESIAN_POINT('Ctrl Pts',(18.360615531112,-16.8680791859056,-1.46447480585023));
#88921=CARTESIAN_POINT('Ctrl Pts',(18.330871940363,-16.8737176293326,-1.46264402126102));
#88922=CARTESIAN_POINT('Ctrl Pts',(18.3220485566474,-16.8754485662734,-1.46210207030407));
#88923=CARTESIAN_POINT('Ctrl Pts',(18.3068432029953,-16.8785322225203,-1.46117003357844));
#88924=CARTESIAN_POINT('Ctrl Pts',(18.3004560173903,-16.8798583132191,-1.46077910342147));
#88925=CARTESIAN_POINT('Ctrl Pts',(18.2882362840569,-16.8824543158398,-1.46003227046569));
#88926=CARTESIAN_POINT('Ctrl Pts',(18.2824027876492,-16.8837194126042,-1.45967621774577));
#88927=CARTESIAN_POINT('Ctrl Pts',(18.2672434753084,-16.8870741703093,-1.45875214469929));
#88928=CARTESIAN_POINT('Ctrl Pts',(18.2579262536683,-16.8892023540657,-1.45818536421874));
#88929=CARTESIAN_POINT('Ctrl Pts',(18.2261829697846,-16.8966794924995,-1.45625813314305));
#88930=CARTESIAN_POINT('Ctrl Pts',(18.2038295264439,-16.9023317695011,-1.45490743175076));
#88931=CARTESIAN_POINT('Ctrl Pts',(18.013001869802,-16.9539151669752,-1.44342145295145));
#88932=CARTESIAN_POINT('Ctrl Pts',(17.8507181972532,-17.0201611612086,-1.43402845207069));
#88933=CARTESIAN_POINT('Ctrl Pts',(17.6219897127354,-17.1484486544967,-1.4197611584354));
#88934=CARTESIAN_POINT('Ctrl Pts',(17.5483186253048,-17.1960041053664,-1.41496680559605));
#88935=CARTESIAN_POINT('Ctrl Pts',(17.4472435822859,-17.2705158003249,-1.4077984934582));
#88936=CARTESIAN_POINT('Ctrl Pts',(17.4172897233129,-17.2938670632764,-1.4055928155219));
#88937=CARTESIAN_POINT('Ctrl Pts',(17.382131184565,-17.3228292997282,-1.40288267925138));
#88938=CARTESIAN_POINT('Ctrl Pts',(17.3763062231341,-17.32768042889,-1.40242955523674));
#88939=CARTESIAN_POINT('Ctrl Pts',(17.3673067243913,-17.3352575967854,-1.40172284187863));
#88940=CARTESIAN_POINT('Ctrl Pts',(17.3641139356787,-17.3379619961014,-1.40147080842526));
#88941=CARTESIAN_POINT('Ctrl Pts',(17.3582169964193,-17.3429870029163,-1.40100283730267));
#88942=CARTESIAN_POINT('Ctrl Pts',(17.3555106795324,-17.3453049789996,-1.40078709230361));
#88943=CARTESIAN_POINT('Ctrl Pts',(17.3494172706157,-17.3505507470784,-1.40029912782624));
#88944=CARTESIAN_POINT('Ctrl Pts',(17.3460336267236,-17.3534824398855,-1.40002662231347));
#88945=CARTESIAN_POINT('Ctrl Pts',(17.3361072826802,-17.3621382062456,-1.39922271506096));
#88946=CARTESIAN_POINT('Ctrl Pts',(17.3295906039502,-17.3678917919791,-1.39868919181648));
#88947=CARTESIAN_POINT('Ctrl Pts',(17.2837281424468,-17.4088892562776,-1.39489463916299));
#88948=CARTESIAN_POINT('Ctrl Pts',(17.245681420375,-17.445551851493,-1.39153840666891));
#88949=CARTESIAN_POINT('Ctrl Pts',(17.1955076965282,-17.4976576891516,-1.38686501324219));
#88950=CARTESIAN_POINT('Ctrl Pts',(17.1821619048552,-17.5119067326764,-1.38559625225881));
#88951=CARTESIAN_POINT('Ctrl Pts',(17.0704045412418,-17.634585567685,-1.37476374261636));
#88952=CARTESIAN_POINT('Ctrl Pts',(16.9832811504003,-17.7527838577972,-1.36495842800338));
#88953=CARTESIAN_POINT('Ctrl Pts',(16.8777709018671,-17.9322388823302,-1.35150931092586));
#88954=CARTESIAN_POINT('Ctrl Pts',(16.8488256589445,-17.986796377786,-1.34758320257808));
#88955=CARTESIAN_POINT('Ctrl Pts',(16.8063135109703,-18.0761579407601,-1.34141720640087));
#88956=CARTESIAN_POINT('Ctrl Pts',(16.7912114292385,-18.1101880506984,-1.33912754616097));
#88957=CARTESIAN_POINT('Ctrl Pts',(16.7727688572228,-18.1548894141365,-1.33619297516809));
#88958=CARTESIAN_POINT('Ctrl Pts',(16.7686050699074,-18.1652118088877,-1.33552028607714));
#88959=CARTESIAN_POINT('Ctrl Pts',(16.7619671080002,-18.1820494622976,-1.33443092439064));
#88960=CARTESIAN_POINT('Ctrl Pts',(16.7594433952834,-18.1885448446606,-1.33401258755429));
#88961=CARTESIAN_POINT('Ctrl Pts',(16.7546526300679,-18.2010577012257,-1.33321029920873));
#88962=CARTESIAN_POINT('Ctrl Pts',(16.7523808363813,-18.2070732661978,-1.33282619209593));
#88963=CARTESIAN_POINT('Ctrl Pts',(16.7472431548165,-18.2208673482705,-1.33194900658151));
#88964=CARTESIAN_POINT('Ctrl Pts',(16.7443954641745,-18.2286525659721,-1.33145654054589));
#88965=CARTESIAN_POINT('Ctrl Pts',(16.7369541499678,-18.249372590471,-1.33015264909309));
#88966=CARTESIAN_POINT('Ctrl Pts',(16.7324404237938,-18.2623358209321,-1.32934387770879));
#88967=CARTESIAN_POINT('Ctrl Pts',(16.6991412232663,-18.3610510614911,-1.32323611835754));
#88968=CARTESIAN_POINT('Ctrl Pts',(16.6757502479701,-18.448530311514,-1.31812043025284));
#88969=CARTESIAN_POINT('Ctrl Pts',(16.6306361033598,-18.6743412206997,-1.30537418636804));
#88970=CARTESIAN_POINT('Ctrl Pts',(16.6168948152901,-18.8138052075209,-1.29793912209419));
#88971=CARTESIAN_POINT('Ctrl Pts',(16.6170159594122,-18.9738905047867,-1.28909419685754));
#88972=CARTESIAN_POINT('Ctrl Pts',(16.6173229666978,-18.9941773247999,-1.28796711722982));
#88973=CARTESIAN_POINT('Ctrl Pts',(16.6196735818504,-19.0738185473015,-1.28350784889897));
#88974=CARTESIAN_POINT('Ctrl Pts',(16.6239226733544,-19.1330753310935,-1.28011460693867));
#88975=CARTESIAN_POINT('Ctrl Pts',(16.6316702820024,-19.2009553189979,-1.27606205837487));
#88976=CARTESIAN_POINT('Ctrl Pts',(16.6327408137604,-19.2098348694499,-1.27552865093646));
#88977=CARTESIAN_POINT('Ctrl Pts',(16.6344383637595,-19.2232018874069,-1.27472036628638));
#88978=CARTESIAN_POINT('Ctrl Pts',(16.6350235911957,-19.2276946907578,-1.27444778780645));
#88979=CARTESIAN_POINT('Ctrl Pts',(16.6360953416554,-19.2357212874388,-1.2739591405539));
#88980=CARTESIAN_POINT('Ctrl Pts',(16.636576377512,-19.2392557606317,-1.27374338405155));
#88981=CARTESIAN_POINT('Ctrl Pts',(16.6376355523248,-19.2468936662814,-1.27327586526396));
#88982=CARTESIAN_POINT('Ctrl Pts',(16.6382167990403,-19.2509965648376,-1.27302393473658));
#88983=CARTESIAN_POINT('Ctrl Pts',(16.6398690473528,-19.262417879234,-1.27232047861236));
#88984=CARTESIAN_POINT('Ctrl Pts',(16.6409663500989,-19.2697323453013,-1.27186750610077));
#88985=CARTESIAN_POINT('Ctrl Pts',(16.647461038454,-19.3115308720028,-1.26926547983125));
#88986=CARTESIAN_POINT('Ctrl Pts',(16.6536719489209,-19.3458808933004,-1.26707452376865));
#88987=CARTESIAN_POINT('Ctrl Pts',(16.6761041766525,-19.4545296219449,-1.26000955504875));
#88988=CARTESIAN_POINT('Ctrl Pts',(16.6954799615833,-19.5281125873802,-1.25502391782212));
#88989=CARTESIAN_POINT('Ctrl Pts',(16.7271552087958,-19.6265459974599,-1.24820176060518));
#88990=CARTESIAN_POINT('Ctrl Pts',(16.7360405261747,-19.6524246263578,-1.24639313502365));
#88991=CARTESIAN_POINT('Ctrl Pts',(16.7454193881274,-19.6781102878244,-1.24458621709267));
#88992=CARTESIAN_POINT('Origin',(18.734,-18.952,0.));
#88993=CARTESIAN_POINT('',(16.7454194499637,-19.6781104571739,-0.444429617385103));
#88994=CARTESIAN_POINT('',(16.7454194499637,-19.6781104571739,-0.666446448202515));
#88995=CARTESIAN_POINT('',(16.7454194499637,-19.6781104571739,0.));
#88996=CARTESIAN_POINT('',(20.3539256943887,-17.5890877707427,0.));
#88997=CARTESIAN_POINT('Ctrl Pts',(16.7454194499637,-19.6781104571739,-0.444429617385103));
#88998=CARTESIAN_POINT('Ctrl Pts',(16.770110945612,-19.7457324388056,-0.440115253521716));
#88999=CARTESIAN_POINT('Ctrl Pts',(16.798260129574,-19.8121054314175,-0.43580088965833));
#89000=CARTESIAN_POINT('Ctrl Pts',(16.8297062682848,-19.8768537091617,-0.431486525794943));
#89001=CARTESIAN_POINT('Ctrl Pts',(16.8611790959266,-19.9416569399905,-0.42716850024957));
#89002=CARTESIAN_POINT('Ctrl Pts',(16.895954251445,-20.0048322531576,-0.422850474704197));
#89003=CARTESIAN_POINT('Ctrl Pts',(16.933824202708,-20.0660269740199,-0.418532449158824));
#89004=CARTESIAN_POINT('Ctrl Pts',(16.9717096227299,-20.1272466911221,-0.414212659827284));
#89005=CARTESIAN_POINT('Ctrl Pts',(17.0126920725612,-20.186483796078,-0.409892870495744));
#89006=CARTESIAN_POINT('Ctrl Pts',(17.0565212752466,-20.2434155520202,-0.405573081164204));
#89007=CARTESIAN_POINT('Ctrl Pts',(17.1004272507063,-20.3004470316303,-0.401245725137602));
#89008=CARTESIAN_POINT('Ctrl Pts',(17.1471896150003,-20.3551647188214,-0.396918369111001));
#89009=CARTESIAN_POINT('Ctrl Pts',(17.1965189468866,-20.4072803892437,-0.3925910130844));
#89010=CARTESIAN_POINT('Ctrl Pts',(17.238558447032,-20.4516944660317,-0.388903148737701));
#89011=CARTESIAN_POINT('Ctrl Pts',(17.2824615173146,-20.49421925598,-0.385215284391002));
#89012=CARTESIAN_POINT('Ctrl Pts',(17.328030443818,-20.5346997842577,-0.381527420044303));
#89013=CARTESIAN_POINT('Ctrl Pts',(17.3823195205318,-20.5829267378796,-0.377133839466685));
#89014=CARTESIAN_POINT('Ctrl Pts',(17.4391958931759,-20.628448704409,-0.372740258889068));
#89015=CARTESIAN_POINT('Ctrl Pts',(17.498359246263,-20.6709767094712,-0.368346678311451));
#89016=CARTESIAN_POINT('Ctrl Pts',(17.5574363013708,-20.7134426815229,-0.363959506382193));
#89017=CARTESIAN_POINT('Ctrl Pts',(17.6187933267003,-20.7529230838071,-0.359572334452935));
#89018=CARTESIAN_POINT('Ctrl Pts',(17.6820956518213,-20.7891679951172,-0.355185162523678));
#89019=CARTESIAN_POINT('Ctrl Pts',(17.7453255105041,-20.8253714144342,-0.350803012885832));
#89020=CARTESIAN_POINT('Ctrl Pts',(17.8104958295947,-20.8583464631661,-0.346420863247986));
#89021=CARTESIAN_POINT('Ctrl Pts',(17.8772429582996,-20.8878864562512,-0.342038713610141));
#89022=CARTESIAN_POINT('Ctrl Pts',(17.9439489461201,-20.9174082417899,-0.33765926499503));
#89023=CARTESIAN_POINT('Ctrl Pts',(18.0122293762549,-20.9434989788705,-0.33327981637992));
#89024=CARTESIAN_POINT('Ctrl Pts',(18.081697252437,-20.9659985415888,-0.32890036776481));
#89025=CARTESIAN_POINT('Ctrl Pts',(18.1511450535803,-20.9884916023148,-0.324522184736118));
#89026=CARTESIAN_POINT('Ctrl Pts',(18.2217791621869,-21.0073954011508,-0.320144001707427));
#89027=CARTESIAN_POINT('Ctrl Pts',(18.2931954849953,-21.0225990388174,-0.315765818678735));
#89028=CARTESIAN_POINT('Ctrl Pts',(18.3646145496345,-21.0378032601853,-0.311387467561893));
#89029=CARTESIAN_POINT('Ctrl Pts',(18.4368154173397,-21.0493069401342,-0.30700911644505));
#89030=CARTESIAN_POINT('Ctrl Pts',(18.5093834475756,-21.0570502142175,-0.302630765328207));
#89031=CARTESIAN_POINT('Ctrl Pts',(18.5820274277171,-21.0648015924333,-0.298247831816702));
#89032=CARTESIAN_POINT('Ctrl Pts',(18.6550388584148,-21.0687846559847,-0.293864898305197));
#89033=CARTESIAN_POINT('Ctrl Pts',(18.7279984288039,-21.0689914929312,-0.289481964793691));
#89034=CARTESIAN_POINT('Ctrl Pts',(18.8009983528725,-21.0691984442785,-0.285096607097214));
#89035=CARTESIAN_POINT('Ctrl Pts',(18.8739458788801,-21.0656250338833,-0.280711249400737));
#89036=CARTESIAN_POINT('Ctrl Pts',(18.946424858768,-21.0583154273227,-0.27632589170426));
#89037=CARTESIAN_POINT('Ctrl Pts',(19.0190319251111,-21.0509929030637,-0.271932784106735));
#89038=CARTESIAN_POINT('Ctrl Pts',(19.091168316046,-21.0399210701979,-0.267539676509209));
#89039=CARTESIAN_POINT('Ctrl Pts',(19.1624267103003,-21.0251954934114,-0.263146568911683));
#89040=CARTESIAN_POINT('Ctrl Pts',(19.2099795641009,-21.0153686764113,-0.260214917062078));
#89041=CARTESIAN_POINT('Ctrl Pts',(19.2571416600211,-21.003915800001,-0.257283265212474));
#89042=CARTESIAN_POINT('Ctrl Pts',(19.3037962227791,-20.9908774520571,-0.254351613362869));
#89043=CARTESIAN_POINT('Ctrl Pts',(19.3728933262966,-20.971567184758,-0.250009730396774));
#89044=CARTESIAN_POINT('Ctrl Pts',(19.4411588243116,-20.9486979955926,-0.245667847430679));
#89045=CARTESIAN_POINT('Ctrl Pts',(19.5081940324577,-20.9223584953269,-0.241325964464583));
#89046=CARTESIAN_POINT('Ctrl Pts',(19.5751282952576,-20.8960586585461,-0.236990619747436));
#89047=CARTESIAN_POINT('Ctrl Pts',(19.6408354886486,-20.8662990562217,-0.232655275030289));
#89048=CARTESIAN_POINT('Ctrl Pts',(19.7049304077652,-20.833218526189,-0.228319930313142));
#89049=CARTESIAN_POINT('Ctrl Pts',(19.7689516598175,-20.8001760170412,-0.223989568395299));
#89050=CARTESIAN_POINT('Ctrl Pts',(19.8313638797399,-20.7638203813565,-0.219659206477455));
#89051=CARTESIAN_POINT('Ctrl Pts',(19.8918019327492,-20.7243384791067,-0.215328844559612));
#89052=CARTESIAN_POINT('Ctrl Pts',(19.952202841651,-20.6848808417024,-0.211001144001965));
#89053=CARTESIAN_POINT('Ctrl Pts',(20.0106315769706,-20.6423010159659,-0.206673443444318));
#89054=CARTESIAN_POINT('Ctrl Pts',(20.0667491221407,-20.5968309267013,-0.202345742886671));
#89055=CARTESIAN_POINT('Ctrl Pts',(20.1228516204485,-20.5513730293844,-0.198019202720377));
#89056=CARTESIAN_POINT('Ctrl Pts',(20.1766437747633,-20.5030267163447,-0.193692662554083));
#89057=CARTESIAN_POINT('Ctrl Pts',(20.2278184819436,-20.4520651129214,-0.189366122387789));
#89058=CARTESIAN_POINT('Ctrl Pts',(20.2789971971884,-20.401099518124,-0.18503924336167));
#89059=CARTESIAN_POINT('Ctrl Pts',(20.3275577103422,-20.3475185761416,-0.180712364335552));
#89060=CARTESIAN_POINT('Ctrl Pts',(20.3732300428321,-20.2916319892705,-0.176385485309434));
#89061=CARTESIAN_POINT('Ctrl Pts',(20.4189571873855,-20.2356783320532,-0.172053413529732));
#89062=CARTESIAN_POINT('Ctrl Pts',(20.461788919467,-20.1774138895481,-0.167721341750031));
#89063=CARTESIAN_POINT('Ctrl Pts',(20.5014963977798,-20.11718045119,-0.163389269970329));
#89064=CARTESIAN_POINT('Ctrl Pts',(20.5412283831299,-20.0569098373883,-0.159054524481558));
#89065=CARTESIAN_POINT('Ctrl Pts',(20.5778320305151,-19.994668236685,-0.154719778992786));
#89066=CARTESIAN_POINT('Ctrl Pts',(20.6111241303052,-19.9308227620085,-0.150385033504014));
#89067=CARTESIAN_POINT('Ctrl Pts',(20.6444832806256,-19.8668487020833,-0.146041557806415));
#89068=CARTESIAN_POINT('Ctrl Pts',(20.6745173629453,-19.8012647680478,-0.141698082108817));
#89069=CARTESIAN_POINT('Ctrl Pts',(20.7010912717234,-19.7344582600432,-0.137354606411219));
#89070=CARTESIAN_POINT('Ctrl Pts',(20.721849646991,-19.6822719379232,-0.133961673167958));
#89071=CARTESIAN_POINT('Ctrl Pts',(20.7404975804328,-19.6293400279684,-0.130568739924696));
#89072=CARTESIAN_POINT('Ctrl Pts',(20.7569922863659,-19.5758519129603,-0.127175806681435));
#89073=CARTESIAN_POINT('Ctrl Pts',(20.7789195445138,-19.5047474197739,-0.12266540659273));
#89074=CARTESIAN_POINT('Ctrl Pts',(20.7971288584811,-19.4323721967961,-0.118155006504025));
#89075=CARTESIAN_POINT('Ctrl Pts',(20.8114809541406,-19.3591386559676,-0.113644606415321));
#89076=CARTESIAN_POINT('Ctrl Pts',(20.8265483375802,-19.2822552609233,-0.108909414481349));
#89077=CARTESIAN_POINT('Ctrl Pts',(20.8373637838653,-19.2044262083738,-0.104174222547377));
#89078=CARTESIAN_POINT('Ctrl Pts',(20.8438249724136,-19.1261481719107,-0.0994390306134055));
#89079=CARTESIAN_POINT('Ctrl Pts',(20.8499589701725,-19.0518340891932,-0.0949436260150769));
#89080=CARTESIAN_POINT('Ctrl Pts',(20.852168892667,-18.9771159048155,-0.0904482214167483));
#89081=CARTESIAN_POINT('Ctrl Pts',(20.8504195396485,-18.9024285143068,-0.0859528168184197));
#89082=CARTESIAN_POINT('Ctrl Pts',(20.848671831534,-18.8278113518075,-0.0814616392162973));
#89083=CARTESIAN_POINT('Ctrl Pts',(20.842972258343,-18.7532253737159,-0.0769704616141749));
#89084=CARTESIAN_POINT('Ctrl Pts',(20.833337630623,-18.6791071407126,-0.0724792840120526));
#89085=CARTESIAN_POINT('Ctrl Pts',(20.8237095451823,-18.6050392368129,-0.067991156090602));
#89086=CARTESIAN_POINT('Ctrl Pts',(20.810151776091,-18.5314388917089,-0.0635030281691514));
#89087=CARTESIAN_POINT('Ctrl Pts',(20.7927329926196,-18.4587379346641,-0.0590149002477008));
#89088=CARTESIAN_POINT('Ctrl Pts',(20.775321490724,-18.3860673688074,-0.0545286484988));
#89089=CARTESIAN_POINT('Ctrl Pts',(20.7540522902898,-18.3142958801147,-0.0500423967498992));
#89090=CARTESIAN_POINT('Ctrl Pts',(20.7290449663564,-18.2438442387327,-0.0455561450009983));
#89091=CARTESIAN_POINT('Ctrl Pts',(20.704034536135,-18.1733838461909,-0.0410693359917531));
#89092=CARTESIAN_POINT('Ctrl Pts',(20.6752851982857,-18.1042440551513,-0.0365825269825079));
#89093=CARTESIAN_POINT('Ctrl Pts',(20.6429658444502,-18.0368287566131,-0.0320957179732627));
#89094=CARTESIAN_POINT('Ctrl Pts',(20.610644937254,-17.9694102179022,-0.0276086933151065));
#89095=CARTESIAN_POINT('Ctrl Pts',(20.5747538739462,-17.9037167392705,-0.0231216686569502));
#89096=CARTESIAN_POINT('Ctrl Pts',(20.5355082322583,-17.8401290141812,-0.018634643998794));
#89097=CARTESIAN_POINT('Ctrl Pts',(20.496235508383,-17.7764974091956,-0.0141445229855435));
#89098=CARTESIAN_POINT('Ctrl Pts',(20.4536038273032,-17.7149748381304,-0.00965440197229298));
#89099=CARTESIAN_POINT('Ctrl Pts',(20.4078725225403,-17.6559136686608,-0.0051642809590425));
#89100=CARTESIAN_POINT('Ctrl Pts',(20.3903400101855,-17.6332707397352,-0.003442853972695));
#89101=CARTESIAN_POINT('Ctrl Pts',(20.3723523439628,-17.6109892567414,-0.0017214269863475));
#89102=CARTESIAN_POINT('Ctrl Pts',(20.3539256943887,-17.5890877707427,0.));
#89103=CARTESIAN_POINT('',(17.1140597194292,-17.5891051077268,-2.19245913160046E-7));
#89104=CARTESIAN_POINT('Origin',(18.734,-18.952,0.));
#89105=CARTESIAN_POINT('Ctrl Pts',(17.1140597194292,-17.5891051077268,-2.19245913160046E-7));
#89106=CARTESIAN_POINT('Ctrl Pts',(17.1607064768662,-17.5336606550706,-0.00438522828538202));
#89107=CARTESIAN_POINT('Ctrl Pts',(17.2102946586576,-17.480504861525,-0.00877023732485088));
#89108=CARTESIAN_POINT('Ctrl Pts',(17.2625708870034,-17.42996670029,-0.0131552463643197));
#89109=CARTESIAN_POINT('Ctrl Pts',(17.3147694940964,-17.3795035795757,-0.0175337444157827));
#89110=CARTESIAN_POINT('Ctrl Pts',(17.3696478802626,-17.3316507087744,-0.0219122424672457));
#89111=CARTESIAN_POINT('Ctrl Pts',(17.4269129074635,-17.2867035301411,-0.0262907405187087));
#89112=CARTESIAN_POINT('Ctrl Pts',(17.4841105391579,-17.2418092500747,-0.0306640854931849));
#89113=CARTESIAN_POINT('Ctrl Pts',(17.5436888539644,-17.1998141657853,-0.035037430467661));
#89114=CARTESIAN_POINT('Ctrl Pts',(17.6053196809544,-17.1609752270281,-0.0394107754421372));
#89115=CARTESIAN_POINT('Ctrl Pts',(17.6669115101636,-17.1221608641608,-0.0437813531204912));
#89116=CARTESIAN_POINT('Ctrl Pts',(17.7305528669281,-17.0864989413485,-0.0481519307988453));
#89117=CARTESIAN_POINT('Ctrl Pts',(17.7958856448175,-17.0542037894968,-0.0525225084771994));
#89118=CARTESIAN_POINT('Ctrl Pts',(17.8611987192173,-17.0219183774296,-0.0568917680479496));
#89119=CARTESIAN_POINT('Ctrl Pts',(17.9282017691101,-16.9929979344006,-0.0612610276186998));
#89120=CARTESIAN_POINT('Ctrl Pts',(17.9965125678451,-16.9676106008614,-0.06563028718945));
#89121=CARTESIAN_POINT('Ctrl Pts',(18.0648253874041,-16.9422225162941,-0.0699996760150934));
#89122=CARTESIAN_POINT('Ctrl Pts',(18.1344455789651,-16.9203679149719,-0.0743690648407367));
#89123=CARTESIAN_POINT('Ctrl Pts',(18.20497303869,-16.9021659886208,-0.07873845366638));
#89124=CARTESIAN_POINT('Ctrl Pts',(18.2755722935749,-16.8839455331716,-0.0831122904187012));
#89125=CARTESIAN_POINT('Ctrl Pts',(18.3470801915499,-16.8693852963437,-0.0874861271710225));
#89126=CARTESIAN_POINT('Ctrl Pts',(18.4190844938149,-16.8585537446679,-0.0918599639233437));
#89127=CARTESIAN_POINT('Ctrl Pts',(18.4911286186646,-16.8477162025113,-0.0962362196628439));
#89128=CARTESIAN_POINT('Ctrl Pts',(18.563669213288,-16.8406114978773,-0.100612475402344));
#89129=CARTESIAN_POINT('Ctrl Pts',(18.6362896320945,-16.8372561185799,-0.104988731141844));
#89130=CARTESIAN_POINT('Ctrl Pts',(18.7090341909997,-16.8338950034698,-0.109372467818921));
#89131=CARTESIAN_POINT('Ctrl Pts',(18.7818583632858,-16.8342960068782,-0.113756204495997));
#89132=CARTESIAN_POINT('Ctrl Pts',(18.8543469087348,-16.8384234999513,-0.118139941173074));
#89133=CARTESIAN_POINT('Ctrl Pts',(18.8963550317497,-16.8408154397493,-0.120680377713149));
#89134=CARTESIAN_POINT('Ctrl Pts',(18.9382505435929,-16.8444579003275,-0.123220814253224));
#89135=CARTESIAN_POINT('Ctrl Pts',(18.9799541383555,-16.8493360796775,-0.125761250793299));
#89136=CARTESIAN_POINT('Ctrl Pts',(19.0521147745614,-16.8577768994061,-0.130157023340392));
#89137=CARTESIAN_POINT('Ctrl Pts',(19.1239757332627,-16.8699525193612,-0.134552795887486));
#89138=CARTESIAN_POINT('Ctrl Pts',(19.1951211678868,-16.8858305324764,-0.138948568434579));
#89139=CARTESIAN_POINT('Ctrl Pts',(19.2661637754887,-16.901685596982,-0.143337987739136));
#89140=CARTESIAN_POINT('Ctrl Pts',(19.3364924469684,-16.9212323267426,-0.147727407043693));
#89141=CARTESIAN_POINT('Ctrl Pts',(19.4056976986063,-16.9443866901998,-0.152116826348249));
#89142=CARTESIAN_POINT('Ctrl Pts',(19.4748249321719,-16.967514950742,-0.156501297270644));
#89143=CARTESIAN_POINT('Ctrl Pts',(19.5428308084353,-16.9942426135354,-0.160885768193038));
#89144=CARTESIAN_POINT('Ctrl Pts',(19.6093188916084,-17.0244352571202,-0.165270239115432));
#89145=CARTESIAN_POINT('Ctrl Pts',(19.6757666906329,-17.0546096074276,-0.169652053551584));
#89146=CARTESIAN_POINT('Ctrl Pts',(19.7406980849855,-17.0882445743231,-0.174033867987736));
#89147=CARTESIAN_POINT('Ctrl Pts',(19.8037359157053,-17.1251573492361,-0.178415682423888));
#89148=CARTESIAN_POINT('Ctrl Pts',(19.866756139595,-17.1620598141979,-0.182796272993973));
#89149=CARTESIAN_POINT('Ctrl Pts',(19.9278834356518,-17.2022380266862,-0.187176863564057));
#89150=CARTESIAN_POINT('Ctrl Pts',(19.9867660616866,-17.2454636849201,-0.191557454134142));
#89151=CARTESIAN_POINT('Ctrl Pts',(20.0456514706292,-17.288691386083,-0.195938251739488));
#89152=CARTESIAN_POINT('Ctrl Pts',(20.1022916128047,-17.3349665330802,-0.200319049344834));
#89153=CARTESIAN_POINT('Ctrl Pts',(20.156365861705,-17.3840190194215,-0.204699846950181));
#89154=CARTESIAN_POINT('Ctrl Pts',(20.2104972294524,-17.4331233201017,-0.209085272009689));
#89155=CARTESIAN_POINT('Ctrl Pts',(20.2620569360998,-17.4850104938255,-0.213470697069196));
#89156=CARTESIAN_POINT('Ctrl Pts',(20.3107600562501,-17.5393724039882,-0.217856122128704));
#89157=CARTESIAN_POINT('Ctrl Pts',(20.359490421265,-17.593764724582,-0.222244000425527));
#89158=CARTESIAN_POINT('Ctrl Pts',(20.4053607162012,-17.6506341638863,-0.22663187872235));
#89159=CARTESIAN_POINT('Ctrl Pts',(20.4481270165511,-17.7096403213523,-0.231019757019172));
#89160=CARTESIAN_POINT('Ctrl Pts',(20.4909690532251,-17.7687509748684,-0.235415405961804));
#89161=CARTESIAN_POINT('Ctrl Pts',(20.5306958563841,-17.8300054996603,-0.239811054904435));
#89162=CARTESIAN_POINT('Ctrl Pts',(20.5671077585183,-17.8930359091735,-0.244206703847067));
#89163=CARTESIAN_POINT('Ctrl Pts',(20.5912140801738,-17.9347648834031,-0.247116821722955));
#89164=CARTESIAN_POINT('Ctrl Pts',(20.6138684164928,-17.9772717133338,-0.250026939598844));
#89165=CARTESIAN_POINT('Ctrl Pts',(20.6350244530402,-18.0204448331188,-0.252937057474733));
#89166=CARTESIAN_POINT('Ctrl Pts',(20.6668851000169,-18.0854628493841,-0.257319647668149));
#89167=CARTESIAN_POINT('Ctrl Pts',(20.6954700316101,-18.1522473407963,-0.261702237861565));
#89168=CARTESIAN_POINT('Ctrl Pts',(20.7205801862023,-18.2204344432736,-0.266084828054982));
#89169=CARTESIAN_POINT('Ctrl Pts',(20.7456525615808,-18.2885189555772,-0.270460824469328));
#89170=CARTESIAN_POINT('Ctrl Pts',(20.767260371406,-18.3580014400403,-0.274836820883674));
#89171=CARTESIAN_POINT('Ctrl Pts',(20.7852512326706,-18.4284950998631,-0.27921281729802));
#89172=CARTESIAN_POINT('Ctrl Pts',(20.8032205403917,-18.4989043063546,-0.28358357114905));
#89173=CARTESIAN_POINT('Ctrl Pts',(20.8175813879169,-18.5703218155193,-0.287954325000079));
#89174=CARTESIAN_POINT('Ctrl Pts',(20.8282307190733,-18.642344230976,-0.292325078851108));
#89175=CARTESIAN_POINT('Ctrl Pts',(20.8388731539879,-18.7143200065093,-0.296693002310752));
#89176=CARTESIAN_POINT('Ctrl Pts',(20.845808770299,-18.7868994338195,-0.301060925770397));
#89177=CARTESIAN_POINT('Ctrl Pts',(20.8489855691776,-18.8596688450713,-0.305428849230041));
#89178=CARTESIAN_POINT('Ctrl Pts',(20.8521613662237,-18.9324153078249,-0.309795395225149));
#89179=CARTESIAN_POINT('Ctrl Pts',(20.8515806778355,-19.0053511525545,-0.314161941220256));
#89180=CARTESIAN_POINT('Ctrl Pts',(20.8472434965741,-19.0780592090539,-0.318528487215364));
#89181=CARTESIAN_POINT('Ctrl Pts',(20.8429062422304,-19.1507684906965,-0.32289510678752));
#89182=CARTESIAN_POINT('Ctrl Pts',(20.8348124001615,-19.2232494936619,-0.327261726359677));
#89183=CARTESIAN_POINT('Ctrl Pts',(20.8230139692876,-19.2950883794611,-0.331628345931833));
#89184=CARTESIAN_POINT('Ctrl Pts',(20.8112033262543,-19.3670016232775,-0.335999485245205));
#89185=CARTESIAN_POINT('Ctrl Pts',(20.7956805170945,-19.438270944489,-0.340370624558577));
#89186=CARTESIAN_POINT('Ctrl Pts',(20.7765488721863,-19.5084917831655,-0.344741763871949));
#89187=CARTESIAN_POINT('Ctrl Pts',(20.757406850392,-19.5787507091909,-0.349115274064269));
#89188=CARTESIAN_POINT('Ctrl Pts',(20.7346522472,-19.6479595605984,-0.353488784256589));
#89189=CARTESIAN_POINT('Ctrl Pts',(20.7084377550415,-19.7157306799303,-0.35786229444891));
#89190=CARTESIAN_POINT('Ctrl Pts',(20.682176526986,-19.7836226234244,-0.36224360185205));
#89191=CARTESIAN_POINT('Ctrl Pts',(20.6524432899172,-19.8500712742597,-0.366624909255191));
#89192=CARTESIAN_POINT('Ctrl Pts',(20.6194379320409,-19.914711173936,-0.371006216658332));
#89193=CARTESIAN_POINT('Ctrl Pts',(20.5965704686666,-19.9594963431777,-0.374041765824277));
#89194=CARTESIAN_POINT('Ctrl Pts',(20.5721332694026,-20.0034137682888,-0.377077314990223));
#89195=CARTESIAN_POINT('Ctrl Pts',(20.5462048528608,-20.0463502964169,-0.380112864156168));
#89196=CARTESIAN_POINT('Ctrl Pts',(20.5087129331597,-20.1084355711665,-0.384502201445419));
#89197=CARTESIAN_POINT('Ctrl Pts',(20.4679538690257,-20.1687127167994,-0.38889153873467));
#89198=CARTESIAN_POINT('Ctrl Pts',(20.424127447363,-20.2268169326104,-0.393280876023921));
#89199=CARTESIAN_POINT('Ctrl Pts',(20.3803660122869,-20.2848349904712,-0.397663704726861));
#89200=CARTESIAN_POINT('Ctrl Pts',(20.333546536813,-20.3406861331264,-0.4020465334298));
#89201=CARTESIAN_POINT('Ctrl Pts',(20.2839132740569,-20.3940325387807,-0.40642936213274));
#89202=CARTESIAN_POINT('Ctrl Pts',(20.234338311065,-20.4473162831732,-0.410807042717946));
#89203=CARTESIAN_POINT('Ctrl Pts',(20.181956453283,-20.4981007839427,-0.415184723303152));
#89204=CARTESIAN_POINT('Ctrl Pts',(20.1270525278191,-20.5460808181321,-0.419562403888359));
#89205=CARTESIAN_POINT('Ctrl Pts',(20.0721834146416,-20.5940304301855,-0.423937308769121));
#89206=CARTESIAN_POINT('Ctrl Pts',(20.0147957688626,-20.6391787874444,-0.428312213649883));
#89207=CARTESIAN_POINT('Ctrl Pts',(19.9552106047207,-20.6812581238548,-0.432687118530645));
#89208=CARTESIAN_POINT('Ctrl Pts',(19.8956435930083,-20.72332464093,-0.437060690610635));
#89209=CARTESIAN_POINT('Ctrl Pts',(19.8338807856146,-20.7623237154589,-0.441434262690625));
#89210=CARTESIAN_POINT('Ctrl Pts',(19.7702742054051,-20.7980294610899,-0.445807834770615));
#89211=CARTESIAN_POINT('Ctrl Pts',(19.7066660505843,-20.8337360906338,-0.450181515120482));
#89212=CARTESIAN_POINT('Ctrl Pts',(19.6412144536897,-20.86614899517,-0.454555195470349));
#89213=CARTESIAN_POINT('Ctrl Pts',(19.5742967209257,-20.8950878572009,-0.458928875820215));
#89214=CARTESIAN_POINT('Ctrl Pts',(19.5073097608989,-20.92405665686,-0.463307080799149));
#89215=CARTESIAN_POINT('Ctrl Pts',(19.4388540801552,-20.949544046669,-0.467685285778082));
#89216=CARTESIAN_POINT('Ctrl Pts',(19.3693269154527,-20.9714179137814,-0.472063490757016));
#89217=CARTESIAN_POINT('Ctrl Pts',(19.2997618805805,-20.9933036951876,-0.476444080463784));
#89218=CARTESIAN_POINT('Ctrl Pts',(19.2291246668025,-21.0115719142762,-0.480824670170553));
#89219=CARTESIAN_POINT('Ctrl Pts',(19.1578249890647,-21.0261411183052,-0.485205259877322));
#89220=CARTESIAN_POINT('Ctrl Pts',(19.0863993186969,-21.0407360673641,-0.489593590460845));
#89221=CARTESIAN_POINT('Ctrl Pts',(19.0143093237697,-21.0516188761684,-0.493981921044368));
#89222=CARTESIAN_POINT('Ctrl Pts',(18.9419715779475,-21.0587597923745,-0.498370251627891));
#89223=CARTESIAN_POINT('Ctrl Pts',(18.892967495442,-21.0635972951603,-0.501343058031128));
#89224=CARTESIAN_POINT('Ctrl Pts',(18.843849807491,-21.0667186668706,-0.504315864434365));
#89225=CARTESIAN_POINT('Ctrl Pts',(18.7947475334652,-21.0681282421389,-0.507288670837602));
#89226=CARTESIAN_POINT('Ctrl Pts',(18.7222522711166,-21.0702093581544,-0.511677762471143));
#89227=CARTESIAN_POINT('Ctrl Pts',(18.6495091063873,-21.0685648466706,-0.516066854104684));
#89228=CARTESIAN_POINT('Ctrl Pts',(18.5769328970345,-21.0631653002941,-0.520455945738225));
#89229=CARTESIAN_POINT('Ctrl Pts',(18.5044640538338,-21.0577737417766,-0.524838544336596));
#89230=CARTESIAN_POINT('Ctrl Pts',(18.4321621525778,-21.0486382115291,-0.529221142934967));
#89231=CARTESIAN_POINT('Ctrl Pts',(18.3604434250555,-21.0357812949817,-0.533603741533338));
#89232=CARTESIAN_POINT('Ctrl Pts',(18.2888085422895,-21.0229394091672,-0.537981216533954));
#89233=CARTESIAN_POINT('Ctrl Pts',(18.2177559511464,-21.0063848642472,-0.54235869153457));
#89234=CARTESIAN_POINT('Ctrl Pts',(18.1476964269545,-20.9861920067275,-0.546736166535186));
#89235=CARTESIAN_POINT('Ctrl Pts',(18.0776810830246,-20.966011883033,-0.551110881054696));
#89236=CARTESIAN_POINT('Ctrl Pts',(18.0086580256525,-20.9421981323211,-0.555485595574205));
#89237=CARTESIAN_POINT('Ctrl Pts',(17.9410261110428,-20.9148758013262,-0.559860310093715));
#89238=CARTESIAN_POINT('Ctrl Pts',(17.8734145608305,-20.8875616972581,-0.564233707359007));
#89239=CARTESIAN_POINT('Ctrl Pts',(17.8071937685408,-20.8567412908305,-0.568607104624299));
#89240=CARTESIAN_POINT('Ctrl Pts',(17.742744149092,-20.8225883668089,-0.572980501889591));
#89241=CARTESIAN_POINT('Ctrl Pts',(17.6782926999987,-20.7884344732282,-0.577354023310197));
#89242=CARTESIAN_POINT('Ctrl Pts',(17.6156129486707,-20.7509481017458,-0.581727544730802));
#89243=CARTESIAN_POINT('Ctrl Pts',(17.5550606677985,-20.7103489559778,-0.586101066151407));
#89244=CARTESIAN_POINT('Ctrl Pts',(17.494445385749,-20.6697075691258,-0.590479137970353));
#89245=CARTESIAN_POINT('Ctrl Pts',(17.4359623948806,-20.6259472108894,-0.594857209789298));
#89246=CARTESIAN_POINT('Ctrl Pts',(17.3799377143115,-20.5793304294077,-0.599235281608243));
#89247=CARTESIAN_POINT('Ctrl Pts',(17.3238823352031,-20.5326881044139,-0.603615752377232));
#89248=CARTESIAN_POINT('Ctrl Pts',(17.2702883027459,-20.4831865672914,-0.60799622314622));
#89249=CARTESIAN_POINT('Ctrl Pts',(17.2194457820157,-20.4311262693854,-0.612376693915209));
#89250=CARTESIAN_POINT('Ctrl Pts',(17.1685131321094,-20.3789736835344,-0.616764929999834));
#89251=CARTESIAN_POINT('Ctrl Pts',(17.1203420532452,-20.3242536410107,-0.621153166084459));
#89252=CARTESIAN_POINT('Ctrl Pts',(17.0751829425931,-20.2673003345456,-0.625541402169084));
#89253=CARTESIAN_POINT('Ctrl Pts',(17.0445739735742,-20.228697227267,-0.628515760619068));
#89254=CARTESIAN_POINT('Ctrl Pts',(17.0153478864754,-20.1890687880074,-0.631490119069052));
#89255=CARTESIAN_POINT('Ctrl Pts',(16.987570942693,-20.1485260330615,-0.634464477519036));
#89256=CARTESIAN_POINT('Ctrl Pts',(16.9460065404289,-20.087859338098,-0.638915198666084));
#89257=CARTESIAN_POINT('Ctrl Pts',(16.9075293837875,-20.0249114258276,-0.643365919813133));
#89258=CARTESIAN_POINT('Ctrl Pts',(16.8723941675653,-19.9600241686811,-0.647816640960181));
#89259=CARTESIAN_POINT('Ctrl Pts',(16.8373240479938,-19.8952571311764,-0.652259116048976));
#89260=CARTESIAN_POINT('Ctrl Pts',(16.8055837807463,-19.8285582959246,-0.65670159113777));
#89261=CARTESIAN_POINT('Ctrl Pts',(16.7773849658163,-19.760298588398,-0.661144066226565));
#89262=CARTESIAN_POINT('Ctrl Pts',(16.7661659280022,-19.7331411265748,-0.662911526885215));
#89263=CARTESIAN_POINT('Ctrl Pts',(16.7555069751172,-19.7057369100368,-0.664678987543865));
#89264=CARTESIAN_POINT('Ctrl Pts',(16.7454194499637,-19.6781104571739,-0.666446448202515));
#89265=CARTESIAN_POINT('Origin',(18.734,19.211,0.));
#89266=CARTESIAN_POINT('',(16.7454194502785,18.4848895419639,-21.2464098152238));
#89267=CARTESIAN_POINT('',(16.7454194503473,18.4848895417754,-21.4658225266004));
#89268=CARTESIAN_POINT('',(16.7454194503191,18.4848895418526,0.));
#89269=CARTESIAN_POINT('',(16.617000615865,19.2093852021581,-21.5109437210328));
#89270=CARTESIAN_POINT('Ctrl Pts',(16.7454194503473,18.4848895417754,-21.4658225266004));
#89271=CARTESIAN_POINT('Ctrl Pts',(16.7444837857047,18.4874520231283,-21.4659708484036));
#89272=CARTESIAN_POINT('Ctrl Pts',(16.7435530647692,18.4900163385141,-21.4661192068269));
#89273=CARTESIAN_POINT('Ctrl Pts',(16.7287346786323,18.5310912408272,-21.4684945740052));
#89274=CARTESIAN_POINT('Ctrl Pts',(16.7159623155329,18.5699940118298,-21.4707298273544));
#89275=CARTESIAN_POINT('Ctrl Pts',(16.6989532213983,18.6273640677302,-21.4740349431173));
#89276=CARTESIAN_POINT('Ctrl Pts',(16.6938233211382,18.6455573547552,-21.4750843617813));
#89277=CARTESIAN_POINT('Ctrl Pts',(16.6733049261105,18.7222435064227,-21.4795220655559));
#89278=CARTESIAN_POINT('Ctrl Pts',(16.660184570789,18.7813079897161,-21.4829745480814));
#89279=CARTESIAN_POINT('Ctrl Pts',(16.6480276910104,18.8497652108745,-21.4870987813877));
#89280=CARTESIAN_POINT('Ctrl Pts',(16.6465012109118,18.8586935344976,-21.4876390532542));
#89281=CARTESIAN_POINT('Ctrl Pts',(16.6443057399693,18.8720502176631,-21.4884512204757));
#89282=CARTESIAN_POINT('Ctrl Pts',(16.6435934062264,18.8764714852112,-21.4887207018453));
#89283=CARTESIAN_POINT('Ctrl Pts',(16.6423404486739,18.8844085510691,-21.4892056795517));
#89284=CARTESIAN_POINT('Ctrl Pts',(16.6417946532296,18.8879234771593,-21.4894208785406));
#89285=CARTESIAN_POINT('Ctrl Pts',(16.6407480096736,18.8947777570967,-21.489841359319));
#89286=CARTESIAN_POINT('Ctrl Pts',(16.6402462936361,18.8981169249839,-21.4900465848015));
#89287=CARTESIAN_POINT('Ctrl Pts',(16.6391505510578,18.9055302987083,-21.490503036673));
#89288=CARTESIAN_POINT('Ctrl Pts',(16.6385604188792,18.9096050541868,-21.4907544778999));
#89289=CARTESIAN_POINT('Ctrl Pts',(16.6371205628663,18.9197556620745,-21.4913821743024));
#89290=CARTESIAN_POINT('Ctrl Pts',(16.6362853629232,18.9258334915099,-21.4917592042927));
#89291=CARTESIAN_POINT('Ctrl Pts',(16.6323979093108,18.9550643923089,-21.4935779299754));
#89292=CARTESIAN_POINT('Ctrl Pts',(16.6297026242297,18.9782623033748,-21.495037625376));
#89293=CARTESIAN_POINT('Ctrl Pts',(16.620518749016,19.0706094574266,-21.5009008934511));
#89294=CARTESIAN_POINT('Ctrl Pts',(16.6170514760726,19.1400099214158,-21.50542257889));
#89295=CARTESIAN_POINT('Ctrl Pts',(16.6170005689228,19.209447963039,-21.5099894604535));
#89296=CARTESIAN_POINT('',(20.3539256943888,17.8480877707428,-22.));
#89297=CARTESIAN_POINT('Ctrl Pts',(16.617000615865,19.2093852021581,-21.5109437210328));
#89298=CARTESIAN_POINT('Ctrl Pts',(16.6169439839438,19.283629630336,-21.5154240901546));
#89299=CARTESIAN_POINT('Ctrl Pts',(16.6207979179101,19.3580185411302,-21.5199044592764));
#89300=CARTESIAN_POINT('Ctrl Pts',(16.6285774612815,19.4320993746177,-21.5243848283982));
#89301=CARTESIAN_POINT('Ctrl Pts',(16.6360763258001,19.5035074389758,-21.5287035498749));
#89302=CARTESIAN_POINT('Ctrl Pts',(16.6472223384959,19.5746287285795,-21.5330222713516));
#89303=CARTESIAN_POINT('Ctrl Pts',(16.6619760547724,19.6450573353873,-21.5373409928283));
#89304=CARTESIAN_POINT('Ctrl Pts',(16.6767199425251,19.7154390245761,-21.5416568372905));
#89305=CARTESIAN_POINT('Ctrl Pts',(16.6950666677318,19.7851284610469,-21.5459726817526));
#89306=CARTESIAN_POINT('Ctrl Pts',(16.7169252865665,19.8537274697937,-21.5502885262148));
#89307=CARTESIAN_POINT('Ctrl Pts',(16.73877701468,19.9223048533567,-21.5546030101481));
#89308=CARTESIAN_POINT('Ctrl Pts',(16.7641382890675,19.9897920183359,-21.5589174940814));
#89309=CARTESIAN_POINT('Ctrl Pts',(16.7928681454194,20.05580537589,-21.5632319780147));
#89310=CARTESIAN_POINT('Ctrl Pts',(16.8215990265588,20.1218210881255,-21.5675466158447));
#89311=CARTESIAN_POINT('Ctrl Pts',(16.8536985269025,20.186362434556,-21.5718612536747));
#89312=CARTESIAN_POINT('Ctrl Pts',(16.8889780731175,20.2490669965483,-21.5761758915047));
#89313=CARTESIAN_POINT('Ctrl Pts',(16.9242925085236,20.3118335692998,-21.5804947962326));
#89314=CARTESIAN_POINT('Ctrl Pts',(16.9627930183938,20.3727593011758,-21.5848137009605));
#89315=CARTESIAN_POINT('Ctrl Pts',(17.0042462838075,20.4315085338981,-21.5891326056885));
#89316=CARTESIAN_POINT('Ctrl Pts',(17.0457242048903,20.4902927096252,-21.5934540792245));
#89317=CARTESIAN_POINT('Ctrl Pts',(17.0901580661956,20.546897422732,-21.5977755527606));
#89318=CARTESIAN_POINT('Ctrl Pts',(17.1372743798887,20.6010202495217,-21.6020970262967));
#89319=CARTESIAN_POINT('Ctrl Pts',(17.1844652826668,20.6552287572955,-21.6064253410887));
#89320=CARTESIAN_POINT('Ctrl Pts',(17.2343467602729,20.7069471894049,-21.6107536558806));
#89321=CARTESIAN_POINT('Ctrl Pts',(17.2866094610681,20.7559108802162,-21.6150819706726));
#89322=CARTESIAN_POINT('Ctrl Pts',(17.3002562194486,20.7686962060366,-21.6162121737669));
#89323=CARTESIAN_POINT('Ctrl Pts',(17.3140651710174,20.7812939269501,-21.6173423768613));
#89324=CARTESIAN_POINT('Ctrl Pts',(17.3280304725231,20.7936998097575,-21.6184725799557));
#89325=CARTESIAN_POINT('Ctrl Pts',(17.3823193345552,20.8419265709082,-21.62286614352));
#89326=CARTESIAN_POINT('Ctrl Pts',(17.4391954779977,20.8874483717554,-21.6272597070843));
#89327=CARTESIAN_POINT('Ctrl Pts',(17.4983585908499,20.9299762383447,-21.6316532706486));
#89328=CARTESIAN_POINT('Ctrl Pts',(17.5574354044305,20.9724420709446,-21.6360404254673));
#89329=CARTESIAN_POINT('Ctrl Pts',(17.618792177104,21.011922361068,-21.6404275802861));
#89330=CARTESIAN_POINT('Ctrl Pts',(17.6820942417089,21.0481671877306,-21.6448147351048));
#89331=CARTESIAN_POINT('Ctrl Pts',(17.7453238390215,21.0843705218375,-21.6491968675719));
#89332=CARTESIAN_POINT('Ctrl Pts',(17.8104938888271,21.1173455129229,-21.6535790000389));
#89333=CARTESIAN_POINT('Ctrl Pts',(17.877240743402,21.1468854760118,-21.657961132506));
#89334=CARTESIAN_POINT('Ctrl Pts',(17.9439464566845,21.1764072313176,-21.662340563923));
#89335=CARTESIAN_POINT('Ctrl Pts',(18.0122266074123,21.2024979658372,-21.6667199953401));
#89336=CARTESIAN_POINT('Ctrl Pts',(18.0816942022227,21.2249975536693,-21.6710994267571));
#89337=CARTESIAN_POINT('Ctrl Pts',(18.1511417219742,21.2474906394691,-21.6754775925863));
#89338=CARTESIAN_POINT('Ctrl Pts',(18.2217755472184,21.2663944910457,-21.6798557584155));
#89339=CARTESIAN_POINT('Ctrl Pts',(18.293191587477,21.2815982090809,-21.6842339242447));
#89340=CARTESIAN_POINT('Ctrl Pts',(18.3646103699649,21.2968025109076,-21.6886122581865));
#89341=CARTESIAN_POINT('Ctrl Pts',(18.4368109563363,21.3083062989017,-21.6929905921282));
#89342=CARTESIAN_POINT('Ctrl Pts',(18.5093787087696,21.3160497085641,-21.69736892607));
#89343=CARTESIAN_POINT('Ctrl Pts',(18.5820224137337,21.3238012228122,-21.7017518425644));
#89344=CARTESIAN_POINT('Ctrl Pts',(18.6550335728178,21.3277844496845,-21.7061347590588));
#89345=CARTESIAN_POINT('Ctrl Pts',(18.7279928778285,21.3279914771872,-21.7105176755531));
#89346=CARTESIAN_POINT('Ctrl Pts',(18.8009925375781,21.3281986191995,-21.7149030162955));
#89347=CARTESIAN_POINT('Ctrl Pts',(18.8739398055028,21.3246254266109,-21.7192883570379));
#89348=CARTESIAN_POINT('Ctrl Pts',(18.9464185362625,21.3173160649466,-21.7236736977803));
#89349=CARTESIAN_POINT('Ctrl Pts',(19.0190253583242,21.3099937854836,-21.7280667887137));
#89350=CARTESIAN_POINT('Ctrl Pts',(19.0911615138916,21.2989222240549,-21.7324598796471));
#89351=CARTESIAN_POINT('Ctrl Pts',(19.1624196844616,21.2841969452915,-21.7368529705805));
#89352=CARTESIAN_POINT('Ctrl Pts',(19.2099750592608,21.2743697753681,-21.7397847759327));
#89353=CARTESIAN_POINT('Ctrl Pts',(19.2571396374613,21.2629163751623,-21.7427165812849));
#89354=CARTESIAN_POINT('Ctrl Pts',(19.3037966250894,21.2498773396251,-21.7456483866371));
#89355=CARTESIAN_POINT('Ctrl Pts',(19.3728942477398,21.2305669125471,-21.7499903038977));
#89356=CARTESIAN_POINT('Ctrl Pts',(19.4411602368598,21.2076975140762,-21.7543322211583));
#89357=CARTESIAN_POINT('Ctrl Pts',(19.5081959039851,21.1813577599646,-21.7586741384189));
#89358=CARTESIAN_POINT('Ctrl Pts',(19.5751306276509,21.1550576687074,-21.7630095175459));
#89359=CARTESIAN_POINT('Ctrl Pts',(19.6408382497924,21.1252977672376,-21.7673448966729));
#89360=CARTESIAN_POINT('Ctrl Pts',(19.7049335619748,21.0922168982419,-21.7716802757999));
#89361=CARTESIAN_POINT('Ctrl Pts',(19.7689552079216,21.0591740498597,-21.7760106721746));
#89362=CARTESIAN_POINT('Ctrl Pts',(19.8313677860799,21.0228180350837,-21.7803410685494));
#89363=CARTESIAN_POINT('Ctrl Pts',(19.8918061585171,20.9833357185646,-21.7846714649241));
#89364=CARTESIAN_POINT('Ctrl Pts',(19.9522073873422,20.9438776666937,-21.7889991999671));
#89365=CARTESIAN_POINT('Ctrl Pts',(20.0106364037878,20.9012973912839,-21.79332693501));
#89366=CARTESIAN_POINT('Ctrl Pts',(20.0667541884382,20.8558268216443,-21.797654670053));
#89367=CARTESIAN_POINT('Ctrl Pts',(20.1228569262381,20.8103684440195,-21.8019812447012));
#89368=CARTESIAN_POINT('Ctrl Pts',(20.1766492784224,20.7620216199763,-21.8063078193494));
#89369=CARTESIAN_POINT('Ctrl Pts',(20.2278241391937,20.7110594792081,-21.8106343939976));
#89370=CARTESIAN_POINT('Ctrl Pts',(20.2790030075947,20.6600933474689,-21.8149613074705));
#89371=CARTESIAN_POINT('Ctrl Pts',(20.3275636296709,20.6065118422404,-21.8192882209435));
#89372=CARTESIAN_POINT('Ctrl Pts',(20.3732360242913,20.550624670072,-21.8236151344164));
#89373=CARTESIAN_POINT('Ctrl Pts',(20.4189632278337,20.4946704307904,-21.8279472403796));
#89374=CARTESIAN_POINT('Ctrl Pts',(20.4617949724119,20.436405384436,-21.8322793463428));
#89375=CARTESIAN_POINT('Ctrl Pts',(20.5015024142213,20.3761713246222,-21.836611452306));
#89376=CARTESIAN_POINT('Ctrl Pts',(20.541234362149,20.3159000903411,-21.8409462319015));
#89377=CARTESIAN_POINT('Ctrl Pts',(20.5778379231948,20.253657851612,-21.845281011497));
#89378=CARTESIAN_POINT('Ctrl Pts',(20.6111298851782,20.1898117255995,-21.8496157910926));
#89379=CARTESIAN_POINT('Ctrl Pts',(20.6444888929844,20.1258370215219,-21.8539593003889));
#89380=CARTESIAN_POINT('Ctrl Pts',(20.6745227819993,20.0602524303901,-21.8583028096851));
#89381=CARTESIAN_POINT('Ctrl Pts',(20.7010964440932,19.9934452566384,-21.8626463189814));
#89382=CARTESIAN_POINT('Ctrl Pts',(20.7218525789006,19.9412635626139,-21.8660389437605));
#89383=CARTESIAN_POINT('Ctrl Pts',(20.7404986559915,19.8883364226189,-21.8694315685395));
#89384=CARTESIAN_POINT('Ctrl Pts',(20.7569919001287,19.8348531654274,-21.8728241933186));
#89385=CARTESIAN_POINT('Ctrl Pts',(20.7789190860527,19.7637490627714,-21.8773345682141));
#89386=CARTESIAN_POINT('Ctrl Pts',(20.7971283710036,19.6913742316258,-21.8818449431095));
#89387=CARTESIAN_POINT('Ctrl Pts',(20.8114804792732,19.6181410790364,-21.886355318005));
#89388=CARTESIAN_POINT('Ctrl Pts',(20.8265479701327,19.54125761101,-21.8910905130881));
#89389=CARTESIAN_POINT('Ctrl Pts',(20.8373635164913,19.4634284696821,-21.8958257081712));
#89390=CARTESIAN_POINT('Ctrl Pts',(20.8438247940449,19.3851503328552,-21.9005609032544));
#89391=CARTESIAN_POINT('Ctrl Pts',(20.8499588376022,19.3108366237006,-21.9050562824811));
#89392=CARTESIAN_POINT('Ctrl Pts',(20.8521688454906,19.2361188075755,-21.9095516617078));
#89393=CARTESIAN_POINT('Ctrl Pts',(20.8504196160406,19.1614317759201,-21.9140470409345));
#89394=CARTESIAN_POINT('Ctrl Pts',(20.8486720313618,19.0868149712324,-21.9185381932313));
#89395=CARTESIAN_POINT('Ctrl Pts',(20.8429726196327,19.0122293415783,-21.923029345528));
#89396=CARTESIAN_POINT('Ctrl Pts',(20.8333381899733,18.9381114437731,-21.9275204978248));
#89397=CARTESIAN_POINT('Ctrl Pts',(20.823710302195,18.8640438728158,-21.9320086005809));
#89398=CARTESIAN_POINT('Ctrl Pts',(20.8101527670998,18.7904438474655,-21.9364967033371));
#89399=CARTESIAN_POINT('Ctrl Pts',(20.7927342525461,18.7177431932619,-21.9409848060932));
#89400=CARTESIAN_POINT('Ctrl Pts',(20.7753230186655,18.6450729268217,-21.945471032891));
#89401=CARTESIAN_POINT('Ctrl Pts',(20.7540541207903,18.5733017207355,-21.9499572596887));
#89402=CARTESIAN_POINT('Ctrl Pts',(20.7290471325623,18.502850341485,-21.9544434864864));
#89403=CARTESIAN_POINT('Ctrl Pts',(20.7040370351564,18.432390202848,-21.9589302710673));
#89404=CARTESIAN_POINT('Ctrl Pts',(20.6752880624039,18.3632506455487,-21.9634170556482));
#89405=CARTESIAN_POINT('Ctrl Pts',(20.6429691045691,18.2958355569623,-21.9679038402291));
#89406=CARTESIAN_POINT('Ctrl Pts',(20.6106485910926,18.228417223416,-21.9723908407771));
#89407=CARTESIAN_POINT('Ctrl Pts',(20.5747579519087,18.1627239264085,-21.976877841325));
#89408=CARTESIAN_POINT('Ctrl Pts',(20.5355127633241,18.099136355671,-21.9813648418729));
#89409=CARTESIAN_POINT('Ctrl Pts',(20.4962404866784,18.0355048951203,-21.9858549394666));
#89410=CARTESIAN_POINT('Ctrl Pts',(20.4536092807961,17.9739824418484,-21.9903450370603));
#89411=CARTESIAN_POINT('Ctrl Pts',(20.4078784777144,17.914921359699,-21.994835134654));
#89412=CARTESIAN_POINT('Ctrl Pts',(20.3903440822918,17.892275783879,-21.996556756436));
#89413=CARTESIAN_POINT('Ctrl Pts',(20.3723544291116,17.8699917351007,-21.998278378218));
#89414=CARTESIAN_POINT('Ctrl Pts',(20.3539256943888,17.8480877707428,-22.));
#89415=CARTESIAN_POINT('',(17.1140599594606,17.8481048224249,-21.9999997809097));
#89416=CARTESIAN_POINT('Origin',(18.734,19.211,-22.));
#89417=CARTESIAN_POINT('',(16.6170002905214,19.2098909158485,-21.2890562790225));
#89418=CARTESIAN_POINT('Ctrl Pts',(17.1140599594606,17.8481048224249,-21.9999997809097));
#89419=CARTESIAN_POINT('Ctrl Pts',(17.1607068911252,17.7926601825033,-21.9956147575322));
#89420=CARTESIAN_POINT('Ctrl Pts',(17.2102952620655,17.739504224746,-21.9912297341546));
#89421=CARTESIAN_POINT('Ctrl Pts',(17.2625716911555,17.6889659228745,-21.9868447107771));
#89422=CARTESIAN_POINT('Ctrl Pts',(17.3147705007786,17.6385026597179,-21.9824661982341));
#89423=CARTESIAN_POINT('Ctrl Pts',(17.3696491012488,17.5906496701831,-21.9780876856911));
#89424=CARTESIAN_POINT('Ctrl Pts',(17.4269143514077,17.5457023967939,-21.9737091731481));
#89425=CARTESIAN_POINT('Ctrl Pts',(17.4841122081179,17.5008080202619,-21.9693358135217));
#89426=CARTESIAN_POINT('Ctrl Pts',(17.5436907567674,17.4588128636585,-21.9649624538953));
#89427=CARTESIAN_POINT('Ctrl Pts',(17.605321823504,17.4199738768232,-21.960589094269));
#89428=CARTESIAN_POINT('Ctrl Pts',(17.6669138937314,17.3811594650113,-21.956218501847));
#89429=CARTESIAN_POINT('Ctrl Pts',(17.7305554975065,17.3454975176011,-21.951847909425));
#89430=CARTESIAN_POINT('Ctrl Pts',(17.7958885256649,17.3132023654455,-21.947477317003));
#89431=CARTESIAN_POINT('Ctrl Pts',(17.8612018513836,17.2809169525184,-21.9431080426178));
#89432=CARTESIAN_POINT('Ctrl Pts',(17.9282051559123,17.2519965330214,-21.9387387682326));
#89433=CARTESIAN_POINT('Ctrl Pts',(17.9965162100301,17.2266092472671,-21.9343694938474));
#89434=CARTESIAN_POINT('Ctrl Pts',(18.0648292857548,17.2012212101981,-21.9300000901573));
#89435=CARTESIAN_POINT('Ctrl Pts',(18.1344497342609,17.179366680706,-21.9256306864672));
#89436=CARTESIAN_POINT('Ctrl Pts',(18.2049774492685,17.1611648503313,-21.9212612827771));
#89437=CARTESIAN_POINT('Ctrl Pts',(18.275576959088,17.142944491113,-21.9168874311828));
#89438=CARTESIAN_POINT('Ctrl Pts',(18.3470851103194,17.1283843746466,-21.9125135795885));
#89439=CARTESIAN_POINT('Ctrl Pts',(18.4190896618186,17.1175529672556,-21.9081397279943));
#89440=CARTESIAN_POINT('Ctrl Pts',(18.4911340360637,17.1067155694601,-21.9037634574032));
#89441=CARTESIAN_POINT('Ctrl Pts',(18.5636748760598,17.0996110331389,-21.8993871868121));
#89442=CARTESIAN_POINT('Ctrl Pts',(18.6362955339105,17.0962558458986,-21.895010916221));
#89443=CARTESIAN_POINT('Ctrl Pts',(18.7090403295018,17.0928949233017,-21.8906271648337));
#89444=CARTESIAN_POINT('Ctrl Pts',(18.7818647321215,17.0932961427629,-21.8862434134464));
#89445=CARTESIAN_POINT('Ctrl Pts',(18.8543534992707,17.0974238752263,-21.8818596620591));
#89446=CARTESIAN_POINT('Ctrl Pts',(18.8963594228442,17.0998158211955,-21.879319357775));
#89447=CARTESIAN_POINT('Ctrl Pts',(18.9382527448405,17.103458157136,-21.8767790534908));
#89448=CARTESIAN_POINT('Ctrl Pts',(18.9799541720406,17.1083360836178,-21.8742387492067));
#89449=CARTESIAN_POINT('Ctrl Pts',(19.0521148556278,17.1167769100605,-21.8698429741465));
#89450=CARTESIAN_POINT('Ctrl Pts',(19.1239758590327,17.1289525413789,-21.8654471990862));
#89451=CARTESIAN_POINT('Ctrl Pts',(19.1951213352851,17.1448305698358,-21.861051424026));
#89452=CARTESIAN_POINT('Ctrl Pts',(19.2661639857042,17.1606856499397,-21.8566620021347));
#89453=CARTESIAN_POINT('Ctrl Pts',(19.3364926969102,17.1802323993941,-21.8522725802435));
#89454=CARTESIAN_POINT('Ctrl Pts',(19.4056979848776,17.2033867859791,-21.8478831583522));
#89455=CARTESIAN_POINT('Ctrl Pts',(19.4748252563206,17.2265150701546,-21.8434986847453));
#89456=CARTESIAN_POINT('Ctrl Pts',(19.5428311670215,17.2532427601722,-21.8391142111383));
#89457=CARTESIAN_POINT('Ctrl Pts',(19.6093192809603,17.2834354339272,-21.8347297375313));
#89458=CARTESIAN_POINT('Ctrl Pts',(19.6757671116488,17.3136098148032,-21.8303479203518));
#89459=CARTESIAN_POINT('Ctrl Pts',(19.7406985339571,17.3472448153046,-21.8259661031722));
#89460=CARTESIAN_POINT('Ctrl Pts',(19.8037363887647,17.3841576262434,-21.8215842859927));
#89461=CARTESIAN_POINT('Ctrl Pts',(19.8667566375372,17.4210601276904,-21.8172036926242));
#89462=CARTESIAN_POINT('Ctrl Pts',(19.9278839545639,17.4612383791652,-21.8128230992558));
#89463=CARTESIAN_POINT('Ctrl Pts',(19.9867665975567,17.5044640783018,-21.8084425058873));
#89464=CARTESIAN_POINT('Ctrl Pts',(20.0456520241437,17.5476918208727,-21.8040617054325));
#89465=CARTESIAN_POINT('Ctrl Pts',(20.1022921799,17.5939670112651,-21.7996809049776));
#89466=CARTESIAN_POINT('Ctrl Pts',(20.156366438267,17.6430195424395,-21.7953001045228));
#89467=CARTESIAN_POINT('Ctrl Pts',(20.2104978161903,17.6921238886346,-21.7909146765541));
#89468=CARTESIAN_POINT('Ctrl Pts',(20.2620575288253,17.7440111093862,-21.7865292485854));
#89469=CARTESIAN_POINT('Ctrl Pts',(20.3107606507593,17.7983730675734,-21.7821438206167));
#89470=CARTESIAN_POINT('Ctrl Pts',(20.3594910179605,17.8527654366668,-21.777755939373));
#89471=CARTESIAN_POINT('Ctrl Pts',(20.4053613108282,17.9096349255095,-21.7733680581292));
#89472=CARTESIAN_POINT('Ctrl Pts',(20.4481276048669,17.9686411330726,-21.7689801768854));
#89473=CARTESIAN_POINT('Ctrl Pts',(20.4909696354496,18.0277518370932,-21.7645845249669));
#89474=CARTESIAN_POINT('Ctrl Pts',(20.5306964282269,18.0890064129735,-21.7601888730484));
#89475=CARTESIAN_POINT('Ctrl Pts',(20.56710831572,18.1520368737118,-21.7557932211298));
#89476=CARTESIAN_POINT('Ctrl Pts',(20.5912144042082,18.1937654950115,-21.7528831282617));
#89477=CARTESIAN_POINT('Ctrl Pts',(20.6138685324289,18.2362719576463,-21.7499730353935));
#89478=CARTESIAN_POINT('Ctrl Pts',(20.6350243872034,18.2794446987657,-21.7470629425253));
#89479=CARTESIAN_POINT('Ctrl Pts',(20.6668849874923,18.3444626081263,-21.7426803587599));
#89480=CARTESIAN_POINT('Ctrl Pts',(20.6954698849173,18.4112469909798,-21.7382977749946));
#89481=CARTESIAN_POINT('Ctrl Pts',(20.720580017359,18.4794339847767,-21.7339151912293));
#89482=CARTESIAN_POINT('Ctrl Pts',(20.7456523700338,18.5475183869707,-21.7295392013357));
#89483=CARTESIAN_POINT('Ctrl Pts',(20.7672601692967,18.6170007611369,-21.7251632114421));
#89484=CARTESIAN_POINT('Ctrl Pts',(20.7852510315621,18.6874943118595,-21.7207872215485));
#89485=CARTESIAN_POINT('Ctrl Pts',(20.8032203398046,18.7579034075081,-21.7164164743267));
#89486=CARTESIAN_POINT('Ctrl Pts',(20.8175811995767,18.8293208069692,-21.7120457271049));
#89487=CARTESIAN_POINT('Ctrl Pts',(20.8282305540802,18.9013431151147,-21.7076749798831));
#89488=CARTESIAN_POINT('Ctrl Pts',(20.838873012161,18.9733187822846,-21.7033070631165));
#89489=CARTESIAN_POINT('Ctrl Pts',(20.8458086628383,19.0458981036007,-21.6989391463499));
#89490=CARTESIAN_POINT('Ctrl Pts',(20.848985506631,19.1186674123577,-21.6945712295833));
#89491=CARTESIAN_POINT('Ctrl Pts',(20.8521613485358,19.1914137717031,-21.6902046903359));
#89492=CARTESIAN_POINT('Ctrl Pts',(20.8515807156441,19.2643495165153,-21.6858381510884));
#89493=CARTESIAN_POINT('Ctrl Pts',(20.8472435998573,19.3370574776133,-21.681471611841));
#89494=CARTESIAN_POINT('Ctrl Pts',(20.8429064110345,19.4097666630956,-21.6771049990621));
#89495=CARTESIAN_POINT('Ctrl Pts',(20.8348126445421,19.4822475744202,-21.6727383862833));
#89496=CARTESIAN_POINT('Ctrl Pts',(20.8230142986461,19.5540863740405,-21.6683717735044));
#89497=CARTESIAN_POINT('Ctrl Pts',(20.8112037407264,19.6259995312979,-21.664000641009));
#89498=CARTESIAN_POINT('Ctrl Pts',(20.7956810261304,19.6972687714271,-21.6596295085136));
#89499=CARTESIAN_POINT('Ctrl Pts',(20.7765494845939,19.7674895353779,-21.6552583760183));
#89500=CARTESIAN_POINT('Ctrl Pts',(20.7574075663198,19.8377483862984,-21.6508848726687));
#89501=CARTESIAN_POINT('Ctrl Pts',(20.7346530755002,19.906957168973,-21.6465113693192));
#89502=CARTESIAN_POINT('Ctrl Pts',(20.7084387039386,19.9747282267858,-21.6421378659696));
#89503=CARTESIAN_POINT('Ctrl Pts',(20.6821775964101,20.0426201093875,-21.637756565374));
#89504=CARTESIAN_POINT('Ctrl Pts',(20.6524444880472,20.109068706537,-21.6333752647783));
#89505=CARTESIAN_POINT('Ctrl Pts',(20.6194392664437,20.1737085605479,-21.6289939641826));
#89506=CARTESIAN_POINT('Ctrl Pts',(20.5965714078508,20.2184946570858,-21.6259583547363));
#89507=CARTESIAN_POINT('Ctrl Pts',(20.572133749745,20.2624129761557,-21.6229227452901));
#89508=CARTESIAN_POINT('Ctrl Pts',(20.5462048156797,20.3053503579875,-21.6198871358438));
#89509=CARTESIAN_POINT('Ctrl Pts',(20.5087128685692,20.3674356733592,-21.6154977957915));
#89510=CARTESIAN_POINT('Ctrl Pts',(20.4679537734929,20.4277128557231,-21.6111084557392));
#89511=CARTESIAN_POINT('Ctrl Pts',(20.4241273179606,20.4858171041695,-21.6067191156869));
#89512=CARTESIAN_POINT('Ctrl Pts',(20.3803658487493,20.5438351950362,-21.6023362841933));
#89513=CARTESIAN_POINT('Ctrl Pts',(20.3335463361778,20.5996863665837,-21.5979534526998));
#89514=CARTESIAN_POINT('Ctrl Pts',(20.2839130339366,20.6530327968647,-21.5935706212063));
#89515=CARTESIAN_POINT('Ctrl Pts',(20.2343380311571,20.70631656623,-21.5891929378029));
#89516=CARTESIAN_POINT('Ctrl Pts',(20.1819561311663,20.7571010876826,-21.5848152543996));
#89517=CARTESIAN_POINT('Ctrl Pts',(20.1270521616165,20.8050811381531,-21.5804375709962));
#89518=CARTESIAN_POINT('Ctrl Pts',(20.0721830041647,20.8530307666663,-21.5760626632818));
#89519=CARTESIAN_POINT('Ctrl Pts',(20.0147953122166,20.8981791359674,-21.5716877555675));
#89520=CARTESIAN_POINT('Ctrl Pts',(19.9552101005245,20.9402584799205,-21.5673128478531));
#89521=CARTESIAN_POINT('Ctrl Pts',(19.8956430411106,20.9823250046532,-21.5629392729282));
#89522=CARTESIAN_POINT('Ctrl Pts',(19.8338801846224,21.0213240823263,-21.5585656980033));
#89523=CARTESIAN_POINT('Ctrl Pts',(19.7702735544122,21.0570298265266,-21.5541921230784));
#89524=CARTESIAN_POINT('Ctrl Pts',(19.7066653494861,21.0927364546977,-21.5498184398764));
#89525=CARTESIAN_POINT('Ctrl Pts',(19.6412137015734,21.1251493532758,-21.5454447566744));
#89526=CARTESIAN_POINT('Ctrl Pts',(19.574295917344,21.154088204713,-21.5410710734725));
#89527=CARTESIAN_POINT('Ctrl Pts',(19.5073089059773,21.1830569936903,-21.5366928656502));
#89528=CARTESIAN_POINT('Ctrl Pts',(19.4388531734526,21.2085443681914,-21.5323146578279));
#89529=CARTESIAN_POINT('Ctrl Pts',(19.3693259569769,21.2304182153262,-21.5279364500056));
#89530=CARTESIAN_POINT('Ctrl Pts',(19.2997608703362,21.2523039767335,-21.523555857456));
#89531=CARTESIAN_POINT('Ctrl Pts',(19.2291236047978,21.270572171152,-21.5191752649063));
#89532=CARTESIAN_POINT('Ctrl Pts',(19.1578238757517,21.2851413457966,-21.5147946723567));
#89533=CARTESIAN_POINT('Ctrl Pts',(19.086398154594,21.2997362652946,-21.5104063389627));
#89534=CARTESIAN_POINT('Ctrl Pts',(19.0143081093411,21.3106190398704,-21.5060180055687));
#89535=CARTESIAN_POINT('Ctrl Pts',(18.9419703140981,21.3177599171367,-21.5016296721748));
#89536=CARTESIAN_POINT('Ctrl Pts',(18.8929666481794,21.3225973491147,-21.4986568911707));
#89537=CARTESIAN_POINT('Ctrl Pts',(18.8438493793155,21.3257186793944,-21.4956841101665));
#89538=CARTESIAN_POINT('Ctrl Pts',(18.7947475234683,21.3271282424259,-21.4927113291624));
#89539=CARTESIAN_POINT('Ctrl Pts',(18.7222522479351,21.3292093584771,-21.4883222368506));
#89540=CARTESIAN_POINT('Ctrl Pts',(18.6495090705527,21.3275648456576,-21.4839331445389));
#89541=CARTESIAN_POINT('Ctrl Pts',(18.576932849213,21.3221652967363,-21.4795440522271));
#89542=CARTESIAN_POINT('Ctrl Pts',(18.5044639937146,21.3167737356532,-21.4751614529316));
#89543=CARTESIAN_POINT('Ctrl Pts',(18.4321620808264,21.3076382016009,-21.4707788536361));
#89544=CARTESIAN_POINT('Ctrl Pts',(18.3604433424476,21.2947812801727,-21.4663962543406));
#89545=CARTESIAN_POINT('Ctrl Pts',(18.2888084484159,21.2819393894075,-21.4620187786179));
#89546=CARTESIAN_POINT('Ctrl Pts',(18.2177558467876,21.2653848384199,-21.4576413028952));
#89547=CARTESIAN_POINT('Ctrl Pts',(18.1476963129808,21.2451919738775,-21.4532638271725));
#89548=CARTESIAN_POINT('Ctrl Pts',(18.0776809591945,21.2250118430934,-21.4488891119159));
#89549=CARTESIAN_POINT('Ctrl Pts',(18.0086578928418,21.2011980843124,-21.4445143966593));
#89550=CARTESIAN_POINT('Ctrl Pts',(17.9410259701971,21.1738757444266,-21.4401396814027));
#89551=CARTESIAN_POINT('Ctrl Pts',(17.8734144117325,21.1465616313814,-21.4357662833863));
#89552=CARTESIAN_POINT('Ctrl Pts',(17.8071936121441,21.1157412151327,-21.43139288537));
#89553=CARTESIAN_POINT('Ctrl Pts',(17.7427439864028,21.0815882805972,-21.4270194873536));
#89554=CARTESIAN_POINT('Ctrl Pts',(17.6782925308258,21.0474343764011,-21.4226459651689));
#89555=CARTESIAN_POINT('Ctrl Pts',(17.6156127740304,21.0099479935908,-21.4182724429842));
#89556=CARTESIAN_POINT('Ctrl Pts',(17.5550604887456,20.9693488359262,-21.4138989207996));
#89557=CARTESIAN_POINT('Ctrl Pts',(17.4944452020835,20.9287074370344,-21.4095208482016));
#89558=CARTESIAN_POINT('Ctrl Pts',(17.4359622076729,20.8849470661681,-21.4051427756037));
#89559=CARTESIAN_POINT('Ctrl Pts',(17.3799375246599,20.8383302716031,-21.4007647030058));
#89560=CARTESIAN_POINT('Ctrl Pts',(17.3238821429895,20.7916879334218,-21.3963842314483));
#89561=CARTESIAN_POINT('Ctrl Pts',(17.2702881090797,20.742186382646,-21.3920037598908));
#89562=CARTESIAN_POINT('Ctrl Pts',(17.2194455880259,20.6901260707491,-21.3876232883333));
#89563=CARTESIAN_POINT('Ctrl Pts',(17.1685129377324,20.637973470818,-21.3832350514533));
#89564=CARTESIAN_POINT('Ctrl Pts',(17.1203418596204,20.5832534138692,-21.3788468145733));
#89565=CARTESIAN_POINT('Ctrl Pts',(17.0751827508733,20.5263000927544,-21.3744585776934));
#89566=CARTESIAN_POINT('Ctrl Pts',(17.0445738577713,20.4876970696618,-21.3714842259559));
#89567=CARTESIAN_POINT('Ctrl Pts',(17.0153478403718,20.4480687194866,-21.3685098742184));
#89568=CARTESIAN_POINT('Ctrl Pts',(16.9875709596013,20.4075260577406,-21.3655355224809));
#89569=CARTESIAN_POINT('Ctrl Pts',(16.9460128341117,20.3468685260888,-21.3610854733995));
#89570=CARTESIAN_POINT('Ctrl Pts',(16.9075410202164,20.283930466216,-21.3566354243181));
#89571=CARTESIAN_POINT('Ctrl Pts',(16.872410100661,20.2190535931582,-21.3521853752368));
#89572=CARTESIAN_POINT('Ctrl Pts',(16.8373354740495,20.1542806772475,-21.3477424568074));
#89573=CARTESIAN_POINT('Ctrl Pts',(16.8055913293712,20.087575522894,-21.3432995383781));
#89574=CARTESIAN_POINT('Ctrl Pts',(16.777389334652,20.0193091637773,-21.3388566199487));
#89575=CARTESIAN_POINT('Ctrl Pts',(16.7492306455235,19.9511476311114,-21.3344205238456));
#89576=CARTESIAN_POINT('Ctrl Pts',(16.7246034665895,19.8814300877347,-21.3299844277425));
#89577=CARTESIAN_POINT('Ctrl Pts',(16.7036730262164,19.8105509815909,-21.3255483316393));
#89578=CARTESIAN_POINT('Ctrl Pts',(16.6827615749465,19.739736180385,-21.3211162601762));
#89579=CARTESIAN_POINT('Ctrl Pts',(16.6655403322362,19.6677623532215,-21.316684188713));
#89580=CARTESIAN_POINT('Ctrl Pts',(16.6521256152427,19.5950417244147,-21.3122521172498));
#89581=CARTESIAN_POINT('Ctrl Pts',(16.6387184405169,19.5223619819308,-21.307822537667));
#89582=CARTESIAN_POINT('Ctrl Pts',(16.6291136261334,19.4489367276423,-21.3033929580842));
#89583=CARTESIAN_POINT('Ctrl Pts',(16.6233766950828,19.3751897217871,-21.2989633785014));
#89584=CARTESIAN_POINT('Ctrl Pts',(16.6190996641549,19.3202094157473,-21.2956610120084));
#89585=CARTESIAN_POINT('Ctrl Pts',(16.6169713926914,19.2650505695404,-21.2923586455155));
#89586=CARTESIAN_POINT('Ctrl Pts',(16.6170002905214,19.2098909158485,-21.2890562790225));
#89587=CARTESIAN_POINT('Ctrl Pts',(16.6170002427963,19.2099860969743,-21.2873807964582));
#89588=CARTESIAN_POINT('Ctrl Pts',(16.6170353690335,19.136643544728,-21.2832143048811));
#89589=CARTESIAN_POINT('Ctrl Pts',(16.6208818290681,19.0633472797757,-21.2791524291455));
#89590=CARTESIAN_POINT('Ctrl Pts',(16.6454751492164,18.828628323952,-21.2662360119634));
#89591=CARTESIAN_POINT('Ctrl Pts',(16.6810081481163,18.6693758580667,-21.257641722875));
#89592=CARTESIAN_POINT('Ctrl Pts',(16.7380003564599,18.5054548669163,-21.24767578307));
#89593=CARTESIAN_POINT('Ctrl Pts',(16.7416702055317,18.4951575047746,-21.2470446570357));
#89594=CARTESIAN_POINT('Ctrl Pts',(16.7454194502785,18.4848895419639,-21.2464098152238));
#89595=CARTESIAN_POINT('Origin',(18.734,19.211,0.));
#89596=CARTESIAN_POINT('',(16.7454193207648,18.4848898966599,-20.4442392307736));
#89597=CARTESIAN_POINT('',(16.7454194503208,18.4848895418481,-20.6683679253911));
#89598=CARTESIAN_POINT('',(16.7454194503191,18.4848895418526,0.));
#89599=CARTESIAN_POINT('Ctrl Pts',(16.7454194503208,18.4848895418481,-20.6683679253911));
#89600=CARTESIAN_POINT('Ctrl Pts',(16.7441348059686,18.4884077652029,-20.6685903690978));
#89601=CARTESIAN_POINT('Ctrl Pts',(16.7428594915517,18.4919294163847,-20.6688125036898));
#89602=CARTESIAN_POINT('Ctrl Pts',(16.7369541254702,18.5083726599832,-20.6698472613802));
#89603=CARTESIAN_POINT('Ctrl Pts',(16.7324403978101,18.5213358962243,-20.6706560331205));
#89604=CARTESIAN_POINT('Ctrl Pts',(16.6991411766923,18.6200512110015,-20.6767637970217));
#89605=CARTESIAN_POINT('Ctrl Pts',(16.6757501909395,18.7075305319096,-20.6818794890831));
#89606=CARTESIAN_POINT('Ctrl Pts',(16.6306360838819,18.9333414187323,-20.6946257313365));
#89607=CARTESIAN_POINT('Ctrl Pts',(16.6168948154794,19.0728053060284,-20.7020607908923));
#89608=CARTESIAN_POINT('Ctrl Pts',(16.617015959299,19.2328903772826,-20.7109057039679));
#89609=CARTESIAN_POINT('Ctrl Pts',(16.617322962857,19.253177071559,-20.7120327766097));
#89610=CARTESIAN_POINT('Ctrl Pts',(16.6196735634269,19.3328182834745,-20.716492044051));
#89611=CARTESIAN_POINT('Ctrl Pts',(16.6239226573551,19.3920751822671,-20.7198852923422));
#89612=CARTESIAN_POINT('Ctrl Pts',(16.6316702786931,19.4599552913066,-20.7239378480795));
#89613=CARTESIAN_POINT('Ctrl Pts',(16.6327408111966,19.4688348488019,-20.7244712559343));
#89614=CARTESIAN_POINT('Ctrl Pts',(16.6344383623655,19.4822018766633,-20.725279541175));
#89615=CARTESIAN_POINT('Ctrl Pts',(16.6350235901553,19.4866946828842,-20.7255521198264));
#89616=CARTESIAN_POINT('Ctrl Pts',(16.6360953412416,19.4947212844047,-20.7260407673693));
#89617=CARTESIAN_POINT('Ctrl Pts',(16.6365763773629,19.4982557595681,-20.7262565239901));
#89618=CARTESIAN_POINT('Ctrl Pts',(16.6376355527491,19.5058936693281,-20.7267240430256));
#89619=CARTESIAN_POINT('Ctrl Pts',(16.638216799776,19.5099965700238,-20.7269759736824));
#89620=CARTESIAN_POINT('Ctrl Pts',(16.6398690489288,19.5214178899476,-20.7276794301417));
#89621=CARTESIAN_POINT('Ctrl Pts',(16.640966352227,19.5287323593995,-20.7281324028595));
#89622=CARTESIAN_POINT('Ctrl Pts',(16.6474610431044,19.5705309000328,-20.7307344299766));
#89623=CARTESIAN_POINT('Ctrl Pts',(16.6536719560285,19.6048809317908,-20.7329253866801));
#89624=CARTESIAN_POINT('Ctrl Pts',(16.6761041950024,19.7135297019645,-20.7399903579684));
#89625=CARTESIAN_POINT('Ctrl Pts',(16.6954799915677,19.787112697731,-20.7449759971092));
#89626=CARTESIAN_POINT('Ctrl Pts',(16.7775784075566,20.0422401502929,-20.7626581998136));
#89627=CARTESIAN_POINT('Ctrl Pts',(16.8609882667792,20.2161881709999,-20.775336111035));
#89628=CARTESIAN_POINT('Ctrl Pts',(16.9785112285705,20.3943876233088,-20.7884543683585));
#89629=CARTESIAN_POINT('Ctrl Pts',(16.9905653835143,20.4120757196994,-20.789759589673));
#89630=CARTESIAN_POINT('Ctrl Pts',(17.007689957475,20.4364029080444,-20.7915596447329));
#89631=CARTESIAN_POINT('Ctrl Pts',(17.0125342137028,20.443198928621,-20.7920630537977));
#89632=CARTESIAN_POINT('Ctrl Pts',(17.0209583857816,20.4548705764766,-20.7929286275569));
#89633=CARTESIAN_POINT('Ctrl Pts',(17.0245192153128,20.4597597971723,-20.7932915220664));
#89634=CARTESIAN_POINT('Ctrl Pts',(17.0319298852457,20.4698439663237,-20.7940406732722));
#89635=CARTESIAN_POINT('Ctrl Pts',(17.0357826741008,20.4750366776866,-20.7944268101332));
#89636=CARTESIAN_POINT('Ctrl Pts',(17.0448502079774,20.4871414292851,-20.7953278534073));
#89637=CARTESIAN_POINT('Ctrl Pts',(17.0500837117351,20.4940393232245,-20.7958420189095));
#89638=CARTESIAN_POINT('Ctrl Pts',(17.0671665107623,20.516270324212,-20.7975015757596));
#89639=CARTESIAN_POINT('Ctrl Pts',(17.0791842625905,20.5314731773975,-20.7986403046101));
#89640=CARTESIAN_POINT('Ctrl Pts',(17.1414400752355,20.6080438292411,-20.8043989483798));
#89641=CARTESIAN_POINT('Ctrl Pts',(17.1948920375782,20.6667222325826,-20.8088862591104));
#89642=CARTESIAN_POINT('Ctrl Pts',(17.367930989628,20.8364655078474,-20.822334799419));
#89643=CARTESIAN_POINT('Ctrl Pts',(17.497141287945,20.9368208092079,-20.8309358220121));
#89644=CARTESIAN_POINT('Ctrl Pts',(17.688822419663,21.0530165625757,-20.8434650797091));
#89645=CARTESIAN_POINT('Ctrl Pts',(17.7424061819017,21.082406269016,-20.8469515340758));
#89646=CARTESIAN_POINT('Ctrl Pts',(17.8053528288565,21.1134685269262,-20.851114699853));
#89647=CARTESIAN_POINT('Ctrl Pts',(17.8135516410907,21.1174487604598,-20.8516582382615));
#89648=CARTESIAN_POINT('Ctrl Pts',(17.8258412984466,21.1233171992305,-20.8524752689664));
#89649=CARTESIAN_POINT('Ctrl Pts',(17.8299130095316,21.1252455460269,-20.8527463345065));
#89650=CARTESIAN_POINT('Ctrl Pts',(17.8372191560455,21.1286771989755,-20.8532334482917));
#89651=CARTESIAN_POINT('Ctrl Pts',(17.8404512609448,21.1301853407614,-20.8534491934587));
#89652=CARTESIAN_POINT('Ctrl Pts',(17.8474673905303,21.1334375913452,-20.8539180889718));
#89653=CARTESIAN_POINT('Ctrl Pts',(17.8512527076603,21.1351786760712,-20.8541714152487));
#89654=CARTESIAN_POINT('Ctrl Pts',(17.8618589949822,21.1400192326833,-20.8548821489742));
#89655=CARTESIAN_POINT('Ctrl Pts',(17.8686912367068,21.1430936501654,-20.8553410489826));
#89656=CARTESIAN_POINT('Ctrl Pts',(17.9088201111944,21.1608955664536,-20.8580419950941));
#89657=CARTESIAN_POINT('Ctrl Pts',(17.94247377324,21.1747974521252,-20.8603296315244));
#89658=CARTESIAN_POINT('Ctrl Pts',(18.0526120484764,21.2170032460245,-20.8678505622547));
#89659=CARTESIAN_POINT('Ctrl Pts',(18.1303749387868,21.2417569011278,-20.8732106832107));
#89660=CARTESIAN_POINT('Ctrl Pts',(18.3869083829587,21.3073779180171,-20.8906947603445));
#89661=CARTESIAN_POINT('Ctrl Pts',(18.5696370348791,21.329557146948,-20.9027594061845));
#89662=CARTESIAN_POINT('Ctrl Pts',(18.775275819617,21.3277152085025,-20.9154088485089));
#89663=CARTESIAN_POINT('Ctrl Pts',(18.7975861840113,21.3271625231044,-20.9167705151485));
#89664=CARTESIAN_POINT('Ctrl Pts',(18.8283705348903,21.325912607305,-20.918635213115));
#89665=CARTESIAN_POINT('Ctrl Pts',(18.8368546841449,21.3255169783263,-20.919147639218));
#89666=CARTESIAN_POINT('Ctrl Pts',(18.8514164671393,21.3247500902328,-20.9200246560591));
#89667=CARTESIAN_POINT('Ctrl Pts',(18.8574952526452,21.3244036515755,-20.9203900205261));
#89668=CARTESIAN_POINT('Ctrl Pts',(18.8700078158497,21.3236363726226,-20.9211405841342));
#89669=CARTESIAN_POINT('Ctrl Pts',(18.8764413407258,21.3232123555106,-20.9215256795733));
#89670=CARTESIAN_POINT('Ctrl Pts',(18.8913808605135,21.3221591626785,-20.9224180679941));
#89671=CARTESIAN_POINT('Ctrl Pts',(18.8998852281543,21.3215079577544,-20.9229246643069));
#89672=CARTESIAN_POINT('Ctrl Pts',(18.9269819601036,21.3192682830074,-20.924534489904));
#89673=CARTESIAN_POINT('Ctrl Pts',(18.9455576820423,21.3174853596041,-20.9256316137445));
#89674=CARTESIAN_POINT('Ctrl Pts',(19.1238298334764,21.2979925299181,-20.9361046018898));
#89675=CARTESIAN_POINT('Ctrl Pts',(19.2810475931405,21.2624024994584,-20.944851978839));
#89676=CARTESIAN_POINT('Ctrl Pts',(19.5595120461599,21.1650354449125,-20.9608717263319));
#89677=CARTESIAN_POINT('Ctrl Pts',(19.6817603834485,21.1087526181623,-20.9681342429073));
#89678=CARTESIAN_POINT('Ctrl Pts',(19.8113926765788,21.0334049665116,-20.9769255568039));
#89679=CARTESIAN_POINT('Ctrl Pts',(19.8248600809897,21.025375675751,-20.9778530679659));
#89680=CARTESIAN_POINT('Ctrl Pts',(19.8431757147607,21.0141782347737,-20.979135784132));
#89681=CARTESIAN_POINT('Ctrl Pts',(19.848102348477,21.0111384579813,-20.9794829513984));
#89682=CARTESIAN_POINT('Ctrl Pts',(19.8559119978043,21.0062754955064,-20.9800367823594));
#89683=CARTESIAN_POINT('Ctrl Pts',(19.8588032234084,21.0044654565429,-20.9802425849317));
#89684=CARTESIAN_POINT('Ctrl Pts',(19.8647631117974,21.0007142146323,-20.9806684349294));
#89685=CARTESIAN_POINT('Ctrl Pts',(19.8678311470892,20.9987721091241,-20.9808885453299));
#89686=CARTESIAN_POINT('Ctrl Pts',(19.8751298005123,20.9941256238551,-20.9814142770803));
#89687=CARTESIAN_POINT('Ctrl Pts',(19.8793558082276,20.9914140763968,-20.9817203715041));
#89688=CARTESIAN_POINT('Ctrl Pts',(19.8935799952022,20.9822157624576,-20.9827562488797));
#89689=CARTESIAN_POINT('Ctrl Pts',(19.9035328190337,20.9756597441554,-20.9834904435821));
#89690=CARTESIAN_POINT('Ctrl Pts',(19.9273113393503,20.9597070902291,-20.9852661621062));
#89691=CARTESIAN_POINT('Ctrl Pts',(19.9410819417546,20.9502301713864,-20.9863123320942));
#89692=CARTESIAN_POINT('Ctrl Pts',(19.9923066907291,20.9140759588294,-20.9902670125705));
#89693=CARTESIAN_POINT('Ctrl Pts',(20.0289987630996,20.886345071146,-20.9932278342395));
#89694=CARTESIAN_POINT('Ctrl Pts',(20.1225691377199,20.8107157722418,-21.0010639092873));
#89695=CARTESIAN_POINT('Ctrl Pts',(20.1778790765798,20.7609766008822,-21.0059869591076));
#89696=CARTESIAN_POINT('Ctrl Pts',(20.3402647246819,20.5986968103234,-21.0211538277651));
#89697=CARTESIAN_POINT('Ctrl Pts',(20.437687782884,20.4771963961483,-21.0312701565337));
#89698=CARTESIAN_POINT('Ctrl Pts',(20.5337906758965,20.3259060871407,-21.0423125560435));
#89699=CARTESIAN_POINT('Ctrl Pts',(20.5462830667372,20.3054826266784,-21.0437748099299));
#89700=CARTESIAN_POINT('Ctrl Pts',(20.5633463681499,20.2764928094153,-21.0458116367639));
#89701=CARTESIAN_POINT('Ctrl Pts',(20.5682085305829,20.268100814879,-21.0463967827793));
#89702=CARTESIAN_POINT('Ctrl Pts',(20.5759804521956,20.2544715625901,-21.0473399793466));
#89703=CARTESIAN_POINT('Ctrl Pts',(20.5789259099059,20.2492549187509,-21.0476993172911));
#89704=CARTESIAN_POINT('Ctrl Pts',(20.5850181695699,20.2383572459213,-21.04844653149));
#89705=CARTESIAN_POINT('Ctrl Pts',(20.588161057374,20.232674091672,-21.0488342642145));
#89706=CARTESIAN_POINT('Ctrl Pts',(20.5955279349209,20.2192069123638,-21.0497485338234));
#89707=CARTESIAN_POINT('Ctrl Pts',(20.5997293508403,20.2114106275309,-21.0502742603779));
#89708=CARTESIAN_POINT('Ctrl Pts',(20.6135045548538,20.1854602837429,-21.0520126115366));
#89709=CARTESIAN_POINT('Ctrl Pts',(20.6228634553418,20.1671930281683,-21.0532176312098));
#89710=CARTESIAN_POINT('Ctrl Pts',(20.6710806053891,20.0696084923807,-21.0595612255425));
#89711=CARTESIAN_POINT('Ctrl Pts',(20.705214565554,19.9880492372561,-21.0645333292169));
#89712=CARTESIAN_POINT('Ctrl Pts',(20.7770398441386,19.7809208602852,-21.0766341031006));
#89713=CARTESIAN_POINT('Ctrl Pts',(20.8083604747271,19.6535480043561,-21.0836115738199));
#89714=CARTESIAN_POINT('Ctrl Pts',(20.8332965312334,19.48679992769,-21.0929118329183));
#89715=CARTESIAN_POINT('Ctrl Pts',(20.83787667287,19.449357379994,-21.0950121627494));
#89716=CARTESIAN_POINT('Ctrl Pts',(20.8458050284077,19.3661528405492,-21.0997434618513));
#89717=CARTESIAN_POINT('Ctrl Pts',(20.848670499354,19.3203658311744,-21.1023896722293));
#89718=CARTESIAN_POINT('Ctrl Pts',(20.8502755330067,19.2669020701046,-21.1055661136968));
#89719=CARTESIAN_POINT('Ctrl Pts',(20.8504631980438,19.2592773280437,-21.1060211745932));
#89720=CARTESIAN_POINT('Ctrl Pts',(20.8506981210273,19.2470456578,-21.1067547148459));
#89721=CARTESIAN_POINT('Ctrl Pts',(20.8507715510948,19.2424392201348,-21.107031768016));
#89722=CARTESIAN_POINT('Ctrl Pts',(20.8508753362342,19.2342515957803,-21.1075256948554));
#89723=CARTESIAN_POINT('Ctrl Pts',(20.8509116410061,19.2306705324151,-21.1077422325706));
#89724=CARTESIAN_POINT('Ctrl Pts',(20.8509695837588,19.223046773013,-21.1082043185131));
#89725=CARTESIAN_POINT('Ctrl Pts',(20.850988728364,19.2190041643376,-21.1084499976598));
#89726=CARTESIAN_POINT('Ctrl Pts',(20.851009275933,19.2080238754976,-21.1091190199955));
#89727=CARTESIAN_POINT('Ctrl Pts',(20.8509881545895,19.2010862745621,-21.1095435926024));
#89728=CARTESIAN_POINT('Ctrl Pts',(20.850706745412,19.1657337806965,-21.1117162145323));
#89729=CARTESIAN_POINT('Ctrl Pts',(20.8499084726236,19.1373275600108,-21.1134918608024));
#89730=CARTESIAN_POINT('Ctrl Pts',(20.8458832247719,19.0539238340679,-21.1187767399629));
#89731=CARTESIAN_POINT('Ctrl Pts',(20.8410811084631,18.9990281919281,-21.1223461858666));
#89732=CARTESIAN_POINT('Ctrl Pts',(20.8165229471249,18.8055808884817,-21.1351170656333));
#89733=CARTESIAN_POINT('Ctrl Pts',(20.785181551683,18.668850858788,-21.1444683302288));
#89734=CARTESIAN_POINT('Ctrl Pts',(20.7117604886859,18.450522780286,-21.1593418081366));
#89735=CARTESIAN_POINT('Ctrl Pts',(20.6774819019281,18.3667583339117,-21.1650403571787));
#89736=CARTESIAN_POINT('Ctrl Pts',(20.631942870125,18.2730818528837,-21.1713957995858));
#89737=CARTESIAN_POINT('Ctrl Pts',(20.6258186638608,18.2607896306808,-21.1722295424608));
#89738=CARTESIAN_POINT('Ctrl Pts',(20.6158043914846,18.2411701042999,-21.1735601263159));
#89739=CARTESIAN_POINT('Ctrl Pts',(20.6119901939496,18.233804713023,-21.1740596096502));
#89740=CARTESIAN_POINT('Ctrl Pts',(20.6051404657361,18.220765807402,-21.1749438456652));
#89741=CARTESIAN_POINT('Ctrl Pts',(20.6021221885951,18.2150833927478,-21.175329201168));
#89742=CARTESIAN_POINT('Ctrl Pts',(20.595778956129,18.2032714937467,-21.1761302720531));
#89743=CARTESIAN_POINT('Ctrl Pts',(20.5924495241137,18.1971444916021,-21.1765458225587));
#89744=CARTESIAN_POINT('Ctrl Pts',(20.5837232567908,18.1812733646736,-21.1776223761956));
#89745=CARTESIAN_POINT('Ctrl Pts',(20.5782796386975,18.1715551040744,-21.1782817014597));
#89746=CARTESIAN_POINT('Ctrl Pts',(20.5542940635624,18.1295163392991,-21.1811348533844));
#89747=CARTESIAN_POINT('Ctrl Pts',(20.5349766564033,18.0976443879412,-21.183300611405));
#89748=CARTESIAN_POINT('Ctrl Pts',(20.4814021730998,18.014297940566,-21.1889868948962));
#89749=CARTESIAN_POINT('Ctrl Pts',(20.4457142261337,17.9637849262658,-21.1924562736943));
#89750=CARTESIAN_POINT('Ctrl Pts',(20.3212210573194,17.8030062838189,-21.2037065296048));
#89751=CARTESIAN_POINT('Ctrl Pts',(20.223580476937,17.7000848238373,-21.2112288528991));
#89752=CARTESIAN_POINT('Ctrl Pts',(20.0589910540881,17.5581737212588,-21.223258989424));
#89753=CARTESIAN_POINT('Ctrl Pts',(19.9989652733674,17.511795401496,-21.2275420500309));
#89754=CARTESIAN_POINT('Ctrl Pts',(19.9287638339729,17.4633390476997,-21.2325973897706));
#89755=CARTESIAN_POINT('Ctrl Pts',(19.920901837859,17.4579901760586,-21.2331641805212));
#89756=CARTESIAN_POINT('Ctrl Pts',(19.9091944341673,17.450139959414,-21.2340095541564));
#89757=CARTESIAN_POINT('Ctrl Pts',(19.9053763767621,17.4475977703068,-21.2342854624305));
#89758=CARTESIAN_POINT('Ctrl Pts',(19.8985631496353,17.4430931889431,-21.2347782479248));
#89759=CARTESIAN_POINT('Ctrl Pts',(19.8955712358379,17.4411259689354,-21.2349947973145));
#89760=CARTESIAN_POINT('Ctrl Pts',(19.8891187543368,17.4369067922628,-21.2354621522842));
#89761=CARTESIAN_POINT('Ctrl Pts',(19.8856566296387,17.4346573942227,-21.2357131168411));
#89762=CARTESIAN_POINT('Ctrl Pts',(19.8760735140468,17.4284708820815,-21.2364082908274));
#89763=CARTESIAN_POINT('Ctrl Pts',(19.869938833672,17.4245552260579,-21.2368538795575));
#89764=CARTESIAN_POINT('Ctrl Pts',(19.8360674586041,17.4031807460777,-21.2393166948758));
#89765=CARTESIAN_POINT('Ctrl Pts',(19.8079500119816,17.3863372265402,-21.2413706024959));
#89766=CARTESIAN_POINT('Ctrl Pts',(19.6371361431522,17.2893284568902,-21.2538526767675));
#89767=CARTESIAN_POINT('Ctrl Pts',(19.4859285474865,17.225280941433,-21.2648702342628));
#89768=CARTESIAN_POINT('Ctrl Pts',(19.2190528685793,17.147143832183,-21.283011092152));
#89769=CARTESIAN_POINT('Ctrl Pts',(19.1068141512045,17.123945737257,-21.2902909633051));
#89770=CARTESIAN_POINT('Ctrl Pts',(18.9790743667114,17.1081849592177,-21.2981493943807));
#89771=CARTESIAN_POINT('Ctrl Pts',(18.9648973957373,17.1065810898969,-21.2990159651469));
#89772=CARTESIAN_POINT('Ctrl Pts',(18.9422909751092,17.1042547815452,-21.3003891248715));
#89773=CARTESIAN_POINT('Ctrl Pts',(18.9338717259411,17.1034393621537,-21.3008986184488));
#89774=CARTESIAN_POINT('Ctrl Pts',(18.9190042014309,17.1020893080248,-21.3017950291876));
#89775=CARTESIAN_POINT('Ctrl Pts',(18.9125579804854,17.1015337380471,-21.3021825985334));
#89776=CARTESIAN_POINT('Ctrl Pts',(18.8992097611272,17.1004449415831,-21.3029829150406));
#89777=CARTESIAN_POINT('Ctrl Pts',(18.8923074835671,17.0999159983141,-21.3033955234339));
#89778=CARTESIAN_POINT('Ctrl Pts',(18.8745622019329,17.0986436410164,-21.3044532160175));
#89779=CARTESIAN_POINT('Ctrl Pts',(18.863715758035,17.0979498470878,-21.3050967408568));
#89780=CARTESIAN_POINT('Ctrl Pts',(18.8182380611991,17.0953923527664,-21.3077829835866));
#89781=CARTESIAN_POINT('Ctrl Pts',(18.7835678675167,17.0942961952269,-21.3098016666494));
#89782=CARTESIAN_POINT('Ctrl Pts',(18.693003011674,17.0936594081099,-21.3150107871875));
#89783=CARTESIAN_POINT('Ctrl Pts',(18.637124974149,17.0954792997746,-21.3181606271481));
#89784=CARTESIAN_POINT('Ctrl Pts',(18.3834491881285,17.1138150099211,-21.3322947095872));
#89785=CARTESIAN_POINT('Ctrl Pts',(18.1885431799121,17.1558775600461,-21.342605255844));
#89786=CARTESIAN_POINT('Ctrl Pts',(17.9724263212463,17.2354715466881,-21.3558294456999));
#89787=CARTESIAN_POINT('Ctrl Pts',(17.9427390876854,17.2471738721778,-21.3576899943198));
#89788=CARTESIAN_POINT('Ctrl Pts',(17.9070441482946,17.2621851007477,-21.3599939118244));
#89789=CARTESIAN_POINT('Ctrl Pts',(17.9007717155182,17.2648586599888,-21.3604013040156));
#89790=CARTESIAN_POINT('Ctrl Pts',(17.8904604959179,17.2693126960198,-21.3610753803084));
#89791=CARTESIAN_POINT('Ctrl Pts',(17.8864141130897,17.2710756084621,-21.3613410179109));
#89792=CARTESIAN_POINT('Ctrl Pts',(17.8791231719682,17.2742792633292,-21.361821717315));
#89793=CARTESIAN_POINT('Ctrl Pts',(17.8758766949128,17.2757155258024,-21.3620365029464));
#89794=CARTESIAN_POINT('Ctrl Pts',(17.8695650932791,17.2785268236595,-21.362455541007));
#89795=CARTESIAN_POINT('Ctrl Pts',(17.8664996722056,17.2799009693586,-21.3626597309355));
#89796=CARTESIAN_POINT('Ctrl Pts',(17.8574560073678,17.2839808797593,-21.3632640922099));
#89797=CARTESIAN_POINT('Ctrl Pts',(17.8514871251231,17.2867071210871,-21.3636655049622));
#89798=CARTESIAN_POINT('Ctrl Pts',(17.8231310026218,17.2998182435485,-21.3655842077487));
#89799=CARTESIAN_POINT('Ctrl Pts',(17.8009148365565,17.3105658416356,-21.3671223586615));
#89800=CARTESIAN_POINT('Ctrl Pts',(17.7387157586516,17.3420096297731,-21.3715176022644));
#89801=CARTESIAN_POINT('Ctrl Pts',(17.699199331507,17.3635956648401,-21.3744154557977));
#89802=CARTESIAN_POINT('Ctrl Pts',(17.578475095543,17.4346308214865,-21.3835372372572));
#89803=CARTESIAN_POINT('Ctrl Pts',(17.4998881911085,17.4883007398057,-21.38986235151));
#89804=CARTESIAN_POINT('Ctrl Pts',(17.3073653770202,17.6397364544719,-21.4060185248264));
#89805=CARTESIAN_POINT('Ctrl Pts',(17.1997103750265,17.7446689067703,-21.4156928981247));
#89806=CARTESIAN_POINT('Ctrl Pts',(17.0950141872719,17.8709947166576,-21.4257089298281));
#89807=CARTESIAN_POINT('Ctrl Pts',(17.0861067058801,17.8819641238075,-21.4265670501198));
#89808=CARTESIAN_POINT('Ctrl Pts',(17.0720934375621,17.899578719601,-21.427926882228));
#89809=CARTESIAN_POINT('Ctrl Pts',(17.0669162429172,17.9061663144287,-21.4284314702998));
#89810=CARTESIAN_POINT('Ctrl Pts',(17.0578483025584,17.917846661631,-21.4293192384057));
#89811=CARTESIAN_POINT('Ctrl Pts',(17.0539413443175,17.9229266386391,-21.4297030642928));
#89812=CARTESIAN_POINT('Ctrl Pts',(17.0459025254215,17.9334778199166,-21.4304956127581));
#89813=CARTESIAN_POINT('Ctrl Pts',(17.041774050096,17.9389515180365,-21.4309041982847));
#89814=CARTESIAN_POINT('Ctrl Pts',(17.0312337451951,17.9530684062924,-21.431951442157));
#89815=CARTESIAN_POINT('Ctrl Pts',(17.0248610484235,17.9617406739723,-21.4325885592966));
#89816=CARTESIAN_POINT('Ctrl Pts',(16.9984529420413,17.9982584079331,-21.4352459079366));
#89817=CARTESIAN_POINT('Ctrl Pts',(16.9790290475874,18.0265410883396,-21.4372424455854));
#89818=CARTESIAN_POINT('Ctrl Pts',(16.9301556403247,18.1015480927593,-21.4423912319857));
#89819=CARTESIAN_POINT('Ctrl Pts',(16.9018312389291,18.148975380904,-21.4455036084188));
#89820=CARTESIAN_POINT('Ctrl Pts',(16.8405503212993,18.2613508687033,-21.4526165738726));
#89821=CARTESIAN_POINT('Ctrl Pts',(16.8090251672351,18.326999033245,-21.4565793428513));
#89822=CARTESIAN_POINT('Ctrl Pts',(16.768406775433,18.4241151244899,-21.4622948417452));
#89823=CARTESIAN_POINT('Ctrl Pts',(16.7565625292272,18.4543722703703,-21.46405612283));
#89824=CARTESIAN_POINT('Ctrl Pts',(16.7454194503473,18.4848895417754,-21.4658225266004));
#89825=CARTESIAN_POINT('Ctrl Pts',(16.7454194502785,18.4848895419639,-21.2464098152238));
#89826=CARTESIAN_POINT('Ctrl Pts',(16.7527638959619,18.4647754922724,-21.245166215107));
#89827=CARTESIAN_POINT('Ctrl Pts',(16.7604130101027,18.4447742578277,-21.243908357521));
#89828=CARTESIAN_POINT('Ctrl Pts',(16.7710464259282,18.4181857438961,-21.2422033215757));
#89829=CARTESIAN_POINT('Ctrl Pts',(16.7737629920154,18.4114926218315,-21.2417712954919));
#89830=CARTESIAN_POINT('Ctrl Pts',(16.778076386766,18.4010193472518,-21.2410906451708));
#89831=CARTESIAN_POINT('Ctrl Pts',(16.7796500728174,18.3972296392127,-21.2408434012105));
#89832=CARTESIAN_POINT('Ctrl Pts',(16.7826138710416,18.3901504835426,-21.240379722062));
#89833=CARTESIAN_POINT('Ctrl Pts',(16.7840012921163,18.3868599684955,-21.2401634505022));
#89834=CARTESIAN_POINT('Ctrl Pts',(16.7871888982541,18.3793531083702,-21.2396683632493));
#89835=CARTESIAN_POINT('Ctrl Pts',(16.7889944540061,18.3751391004608,-21.2393892238339));
#89836=CARTESIAN_POINT('Ctrl Pts',(16.7945891480335,18.3621978617488,-21.2385283034645));
#89837=CARTESIAN_POINT('Ctrl Pts',(16.7984233825829,18.3534904239784,-21.2379438745834));
#89838=CARTESIAN_POINT('Ctrl Pts',(16.8514177160967,18.2353082466656,-21.2299441362284));
#89839=CARTESIAN_POINT('Ctrl Pts',(16.9097358236781,18.1301928946525,-21.2220488041687));
#89840=CARTESIAN_POINT('Ctrl Pts',(17.0373255766414,17.9402392757908,-21.2069315721899));
#89841=CARTESIAN_POINT('Ctrl Pts',(17.1049006033556,17.8546904660381,-21.1997374915614));
#89842=CARTESIAN_POINT('Ctrl Pts',(17.2157140416318,17.7346993717156,-21.1892443898919));
#89843=CARTESIAN_POINT('Ctrl Pts',(17.2542010033776,17.6961232655033,-21.1857967859413));
#89844=CARTESIAN_POINT('Ctrl Pts',(17.3107065019804,17.6436979985561,-21.181006856892));
#89845=CARTESIAN_POINT('Ctrl Pts',(17.3275227324188,17.628589906926,-21.1796131082781));
#89846=CARTESIAN_POINT('Ctrl Pts',(17.3536807704653,17.6058354046499,-21.1774926542392));
#89847=CARTESIAN_POINT('Ctrl Pts',(17.3628509736745,17.5979950680005,-21.176757991135));
#89848=CARTESIAN_POINT('Ctrl Pts',(17.3799856616499,17.5835969800569,-21.1754011419974));
#89849=CARTESIAN_POINT('Ctrl Pts',(17.38793198132,17.5770182642513,-21.1747781082329));
#89850=CARTESIAN_POINT('Ctrl Pts',(17.4010997668257,17.5662779744504,-21.1737557539507));
#89851=CARTESIAN_POINT('Ctrl Pts',(17.406293329267,17.5620826063739,-21.1733550677939));
#89852=CARTESIAN_POINT('Ctrl Pts',(17.4165504002975,17.5538768082451,-21.1725686783795));
#89853=CARTESIAN_POINT('Ctrl Pts',(17.4216125853113,17.5498648472801,-21.1721829161296));
#89854=CARTESIAN_POINT('Ctrl Pts',(17.4333448195624,17.5406537425252,-21.1712942157636));
#89855=CARTESIAN_POINT('Ctrl Pts',(17.4400278479259,17.5354712502974,-21.1707919435669));
#89856=CARTESIAN_POINT('Ctrl Pts',(17.4580877972068,17.5216387894874,-21.1694450867428));
#89857=CARTESIAN_POINT('Ctrl Pts',(17.4695216754146,17.5130636553794,-21.1686034424332));
#89858=CARTESIAN_POINT('Ctrl Pts',(17.5748866282003,17.4356971170166,-21.1609454221046));
#89859=CARTESIAN_POINT('Ctrl Pts',(17.6742615063459,17.3746439131274,-21.154443169733));
#89860=CARTESIAN_POINT('Ctrl Pts',(17.9233755373307,17.2485876644494,-21.1391557000502));
#89861=CARTESIAN_POINT('Ctrl Pts',(18.0765562199388,17.192106719694,-21.1305551663233));
#89862=CARTESIAN_POINT('Ctrl Pts',(18.266459240139,17.1460146277258,-21.1193368266112));
#89863=CARTESIAN_POINT('Ctrl Pts',(18.2984190236616,17.1390376699283,-21.1174292941519));
#89864=CARTESIAN_POINT('Ctrl Pts',(18.3376489249934,17.1314213214243,-21.1150499678368));
#89865=CARTESIAN_POINT('Ctrl Pts',(18.3447792426289,17.1300750004835,-21.1146159886861));
#89866=CARTESIAN_POINT('Ctrl Pts',(18.3559636171692,17.1280227014596,-21.1139326859989));
#89867=CARTESIAN_POINT('Ctrl Pts',(18.3600131283766,17.1272918265339,-21.1136847550195));
#89868=CARTESIAN_POINT('Ctrl Pts',(18.3675825380436,17.1259484398437,-21.1132202884411));
#89869=CARTESIAN_POINT('Ctrl Pts',(18.3711018644598,17.1253330305354,-21.1130039196444));
#89870=CARTESIAN_POINT('Ctrl Pts',(18.3791347787413,17.1239492968614,-21.112509106204));
#89871=CARTESIAN_POINT('Ctrl Pts',(18.3836492936083,17.1231867074972,-21.1122303413077));
#89872=CARTESIAN_POINT('Ctrl Pts',(18.3975214270781,17.1208896943121,-21.111371748493));
#89873=CARTESIAN_POINT('Ctrl Pts',(18.4068867606263,17.1194035186212,-21.1107892932738));
#89874=CARTESIAN_POINT('Ctrl Pts',(18.5359034258415,17.0998176758328,-21.1027298189923));
#89875=CARTESIAN_POINT('Ctrl Pts',(18.6568688960735,17.0919490118058,-21.0947647638725));
#89876=CARTESIAN_POINT('Ctrl Pts',(18.9567054216094,17.0981577753165,-21.0749511707336));
#89877=CARTESIAN_POINT('Ctrl Pts',(19.1344308515458,17.1245244433609,-21.0632060404949));
#89878=CARTESIAN_POINT('Ctrl Pts',(19.3274192740309,17.17875890594,-21.0508913153535));
#89879=CARTESIAN_POINT('Ctrl Pts',(19.3480071303989,17.1848841108301,-21.0495820777288));
#89880=CARTESIAN_POINT('Ctrl Pts',(19.3771084755845,17.1940265418937,-21.0477372462095));
#89881=CARTESIAN_POINT('Ctrl Pts',(19.3857008491468,17.1967863943371,-21.0471932686109));
#89882=CARTESIAN_POINT('Ctrl Pts',(19.4004789189037,17.2016375436408,-21.0462588492245));
#89883=CARTESIAN_POINT('Ctrl Pts',(19.4066730193373,17.203702652593,-21.0458675515026));
#89884=CARTESIAN_POINT('Ctrl Pts',(19.418504608993,17.2077082127442,-21.0451207645081));
#89885=CARTESIAN_POINT('Ctrl Pts',(19.4241436394943,17.2096438841114,-21.04476512172));
#89886=CARTESIAN_POINT('Ctrl Pts',(19.438764144066,17.2147317058771,-21.043843726122));
#89887=CARTESIAN_POINT('Ctrl Pts',(19.4477327341011,17.2179206765278,-21.0432791987971));
#89888=CARTESIAN_POINT('Ctrl Pts',(19.4781302344891,17.2289606422007,-21.0413679003346));
#89889=CARTESIAN_POINT('Ctrl Pts',(19.4994540483372,17.2370977781957,-21.0400306581472));
#89890=CARTESIAN_POINT('Ctrl Pts',(19.6856724696758,17.3116300658952,-21.0283732534292));
#89891=CARTESIAN_POINT('Ctrl Pts',(19.8417242553545,17.3982010041257,-21.0188269506874));
#89892=CARTESIAN_POINT('Ctrl Pts',(20.0540677428375,17.5537694809917,-21.0044991662263));
#89893=CARTESIAN_POINT('Ctrl Pts',(20.1198771180721,17.6083976954555,-20.9998161647084));
#89894=CARTESIAN_POINT('Ctrl Pts',(20.2095008235223,17.6924522552349,-20.9927980021979));
#89895=CARTESIAN_POINT('Ctrl Pts',(20.2361160809054,17.7187745394609,-20.9906232038976));
#89896=CARTESIAN_POINT('Ctrl Pts',(20.2672424102436,17.7512350550082,-20.9879473165036));
#89897=CARTESIAN_POINT('Ctrl Pts',(20.2724377462836,17.7567114178692,-20.9874960708343));
#89898=CARTESIAN_POINT('Ctrl Pts',(20.2804622239475,17.7652610754076,-20.9867916748433));
#89899=CARTESIAN_POINT('Ctrl Pts',(20.2833118054406,17.7683152191111,-20.9865400643781));
#89900=CARTESIAN_POINT('Ctrl Pts',(20.2885758113405,17.7739906932484,-20.9860724860825));
#89901=CARTESIAN_POINT('Ctrl Pts',(20.2909926624724,17.7766096942194,-20.9858567084005));
#89902=CARTESIAN_POINT('Ctrl Pts',(20.2964367537521,17.7825391102994,-20.985368171404));
#89903=CARTESIAN_POINT('Ctrl Pts',(20.2994600745885,17.7858530332306,-20.9850951229519));
#89904=CARTESIAN_POINT('Ctrl Pts',(20.3083387009505,17.7956474163333,-20.9842881671894));
#89905=CARTESIAN_POINT('Ctrl Pts',(20.3141643781015,17.8021544394278,-20.9837521148015));
#89906=CARTESIAN_POINT('Ctrl Pts',(20.3555539695298,17.8489644449988,-20.9798974988602));
#89907=CARTESIAN_POINT('Ctrl Pts',(20.3896088126729,17.890569565895,-20.9764803818685));
#89908=CARTESIAN_POINT('Ctrl Pts',(20.5153598001475,18.056721939522,-20.9630097009873));
#89909=CARTESIAN_POINT('Ctrl Pts',(20.5948898223481,18.1898764151451,-20.952619438118));
#89910=CARTESIAN_POINT('Ctrl Pts',(20.6978949182326,18.4150996133364,-20.9365437916937));
#89911=CARTESIAN_POINT('Ctrl Pts',(20.7309679248523,18.5021532301219,-20.9306407298613));
#89912=CARTESIAN_POINT('Ctrl Pts',(20.7643902908689,18.6112919632435,-20.9236315493787));
#89913=CARTESIAN_POINT('Ctrl Pts',(20.7702684598198,18.6315646949074,-20.9223453074031));
#89914=CARTESIAN_POINT('Ctrl Pts',(20.7782090643501,18.6605650857446,-20.9205270515309));
#89915=CARTESIAN_POINT('Ctrl Pts',(20.780520614879,18.6692226745821,-20.9199869760399));
#89916=CARTESIAN_POINT('Ctrl Pts',(20.7844182317344,18.6842016095812,-20.919057205311));
#89917=CARTESIAN_POINT('Ctrl Pts',(20.7860301923636,18.6905160326393,-20.9186666758591));
#89918=CARTESIAN_POINT('Ctrl Pts',(20.7890639176096,18.7026330225814,-20.9179199534781));
#89919=CARTESIAN_POINT('Ctrl Pts',(20.790490325767,18.7084343522047,-20.9175636138014));
#89920=CARTESIAN_POINT('Ctrl Pts',(20.7941422285357,18.7235628803697,-20.9166373739574));
#89921=CARTESIAN_POINT('Ctrl Pts',(20.7963289592036,18.732899366223,-20.9160687260988));
#89922=CARTESIAN_POINT('Ctrl Pts',(20.8036013484556,18.7649282008543,-20.9141279005866));
#89923=CARTESIAN_POINT('Ctrl Pts',(20.8083766171052,18.7876898241974,-20.9127656655612));
#89924=CARTESIAN_POINT('Ctrl Pts',(20.845241861615,18.9790496212848,-20.9014446205915));
#89925=CARTESIAN_POINT('Ctrl Pts',(20.857096166532,19.1508943033247,-20.8921988796554));
#89926=CARTESIAN_POINT('Ctrl Pts',(20.8433539222923,19.4119216027589,-20.8779848727349));
#89927=CARTESIAN_POINT('Ctrl Pts',(20.8329416094389,19.5011465531038,-20.8730802610273));
#89928=CARTESIAN_POINT('Ctrl Pts',(20.8100173883943,19.62732161828,-20.8657636090026));
#89929=CARTESIAN_POINT('Ctrl Pts',(20.8021016595428,19.6650121064817,-20.8635279366092));
#89930=CARTESIAN_POINT('Ctrl Pts',(20.7913966032449,19.7098648360944,-20.8607845992553));
#89931=CARTESIAN_POINT('Ctrl Pts',(20.7895901366942,19.7172569443252,-20.8603297544147));
#89932=CARTESIAN_POINT('Ctrl Pts',(20.7867272403788,19.7287040025151,-20.8596209541419));
#89933=CARTESIAN_POINT('Ctrl Pts',(20.7856985376896,19.7327659124137,-20.8593685699367));
#89934=CARTESIAN_POINT('Ctrl Pts',(20.7837728184429,19.740276003082,-20.8589002766002));
#89935=CARTESIAN_POINT('Ctrl Pts',(20.7828791535374,19.7437249837284,-20.8586845622513));
#89936=CARTESIAN_POINT('Ctrl Pts',(20.780844840466,19.7514953042835,-20.8581971046279));
#89937=CARTESIAN_POINT('Ctrl Pts',(20.7796992186585,19.7558152722044,-20.8579250779148));
#89938=CARTESIAN_POINT('Ctrl Pts',(20.7762947799886,19.7684907614031,-20.8571239732019));
#89939=CARTESIAN_POINT('Ctrl Pts',(20.7739984209429,19.7768359780909,-20.8565927959621));
#89940=CARTESIAN_POINT('Ctrl Pts',(20.7575867844008,19.8350789705842,-20.8528604802505));
#89941=CARTESIAN_POINT('Ctrl Pts',(20.7416946143209,19.8844533466567,-20.8495675972214));
#89942=CARTESIAN_POINT('Ctrl Pts',(20.7166532929313,19.9534551774318,-20.8448281585302));
#89943=CARTESIAN_POINT('Ctrl Pts',(20.7089898900291,19.9736064913446,-20.843426985138));
#89944=CARTESIAN_POINT('Ctrl Pts',(20.6839297042274,20.0365908746419,-20.8390002873614));
#89945=CARTESIAN_POINT('Ctrl Pts',(20.6654371256026,20.0789726806086,-20.8359523654633));
#89946=CARTESIAN_POINT('Ctrl Pts',(20.5985795303598,20.2194598390507,-20.8256748347791));
#89947=CARTESIAN_POINT('Ctrl Pts',(20.5440021641236,20.3144236286371,-20.8184438758655));
#89948=CARTESIAN_POINT('Ctrl Pts',(20.4512734484407,20.4502311454526,-20.80787401141));
#89949=CARTESIAN_POINT('Ctrl Pts',(20.418454238454,20.4944861381966,-20.8043867236253));
#89950=CARTESIAN_POINT('Ctrl Pts',(20.3624588546783,20.5641395459459,-20.7988317161779));
#89951=CARTESIAN_POINT('Ctrl Pts',(20.3403266230553,20.5903403743556,-20.7967256051754));
#89952=CARTESIAN_POINT('Ctrl Pts',(20.3103939659607,20.624077444834,-20.7939898715823));
#89953=CARTESIAN_POINT('Ctrl Pts',(20.3031594625429,20.6321067478945,-20.7933369267554));
#89954=CARTESIAN_POINT('Ctrl Pts',(20.2912071382511,20.645169624564,-20.7922714823085));
#89955=CARTESIAN_POINT('Ctrl Pts',(20.2865257054468,20.6502360887362,-20.791857453829));
#89956=CARTESIAN_POINT('Ctrl Pts',(20.2774141983572,20.660000796708,-20.7910579020173));
#89957=CARTESIAN_POINT('Ctrl Pts',(20.2729872327527,20.6647018247911,-20.7906722524881));
#89958=CARTESIAN_POINT('Ctrl Pts',(20.2627134855329,20.6755120634761,-20.7897837149294));
#89959=CARTESIAN_POINT('Ctrl Pts',(20.2568514459799,20.6816066712615,-20.7892814932977));
#89960=CARTESIAN_POINT('Ctrl Pts',(20.2409826764744,20.6979083780975,-20.7879345635319));
#89961=CARTESIAN_POINT('Ctrl Pts',(20.2309087190409,20.7080496363955,-20.7870927985867));
#89962=CARTESIAN_POINT('Ctrl Pts',(20.1373585181349,20.8003362920003,-20.7793944137813));
#89963=CARTESIAN_POINT('Ctrl Pts',(20.0472983544054,20.8755292731566,-20.7728560863591));
#89964=CARTESIAN_POINT('Ctrl Pts',(19.81740811117,21.0371351496082,-20.7574736466199));
#89965=CARTESIAN_POINT('Ctrl Pts',(19.6728753792947,21.1154798236972,-20.7488161660152));
#89966=CARTESIAN_POINT('Ctrl Pts',(19.4917871752002,21.1879731076745,-20.7376000975935));
#89967=CARTESIAN_POINT('Ctrl Pts',(19.4625461418193,21.1989346964479,-20.7357770028248));
#89968=CARTESIAN_POINT('Ctrl Pts',(19.4263259160233,21.2116061466475,-20.7334917901452));
#89969=CARTESIAN_POINT('Ctrl Pts',(19.4195648288067,21.2139330967818,-20.7330640753817));
#89970=CARTESIAN_POINT('Ctrl Pts',(19.4089178709198,21.2175372156843,-20.732388550745));
#89971=CARTESIAN_POINT('Ctrl Pts',(19.4050397935629,21.2188374748014,-20.7321420833069));
#89972=CARTESIAN_POINT('Ctrl Pts',(19.3977650548435,21.2212531515996,-20.731678929481));
#89973=CARTESIAN_POINT('Ctrl Pts',(19.3943693280501,21.2223712067753,-20.7314624011407));
#89974=CARTESIAN_POINT('Ctrl Pts',(19.3865863820361,21.2249119359246,-20.7309653635711));
#89975=CARTESIAN_POINT('Ctrl Pts',(19.3821973483342,21.2263288734997,-20.7306845220782));
#89976=CARTESIAN_POINT('Ctrl Pts',(19.3686045105854,21.2306681325474,-20.7298131417432));
#89977=CARTESIAN_POINT('Ctrl Pts',(19.35938546631,21.2335417822388,-20.7292198623444));
#89978=CARTESIAN_POINT('Ctrl Pts',(19.2481026467415,21.2673959472365,-20.7220336719855));
#89979=CARTESIAN_POINT('Ctrl Pts',(19.1438693330105,21.2906796746592,-20.7150597754286));
#89980=CARTESIAN_POINT('Ctrl Pts',(18.9301071896042,21.3217327058625,-20.7008103069896));
#89981=CARTESIAN_POINT('Ctrl Pts',(18.8208111528296,21.3290456101083,-20.6935552862598));
#89982=CARTESIAN_POINT('Ctrl Pts',(18.6488221090727,21.3272123274248,-20.6824362339002));
#89983=CARTESIAN_POINT('Ctrl Pts',(18.586264940794,21.3237672403705,-20.6784512248014));
#89984=CARTESIAN_POINT('Ctrl Pts',(18.4991746404988,21.3150831384411,-20.6729961128224));
#89985=CARTESIAN_POINT('Ctrl Pts',(18.4744463772579,21.3121760521088,-20.6714575296165));
#89986=CARTESIAN_POINT('Ctrl Pts',(18.4312405861266,21.3063223000883,-20.6687868417886));
#89987=CARTESIAN_POINT('Ctrl Pts',(18.4127405147806,21.3035656936721,-20.6676489558615));
#89988=CARTESIAN_POINT('Ctrl Pts',(18.385854476093,21.2991945650397,-20.6660031009818));
#89989=CARTESIAN_POINT('Ctrl Pts',(18.3774382922013,21.2977739693465,-20.6654890158072));
#89990=CARTESIAN_POINT('Ctrl Pts',(18.3626811095882,21.2951911706103,-20.6645895046686));
#89991=CARTESIAN_POINT('Ctrl Pts',(18.3563364422925,21.2940508377454,-20.6642033892572));
#89992=CARTESIAN_POINT('Ctrl Pts',(18.3440146539,21.2917780843284,-20.6634546926165));
#89993=CARTESIAN_POINT('Ctrl Pts',(18.3380370168394,21.2906488462115,-20.6630920142653));
#89994=CARTESIAN_POINT('Ctrl Pts',(18.3237394641117,21.2878840090065,-20.6622257859679));
#89995=CARTESIAN_POINT('Ctrl Pts',(18.3154243029064,21.2862241525087,-20.6617230131681));
#89996=CARTESIAN_POINT('Ctrl Pts',(18.2853398151381,21.2800305668477,-20.6599074352307));
#89997=CARTESIAN_POINT('Ctrl Pts',(18.2636318046011,21.2752037845176,-20.6586039834267));
#89998=CARTESIAN_POINT('Ctrl Pts',(18.0627480670869,21.2272035750021,-20.6465932360829));
#89999=CARTESIAN_POINT('Ctrl Pts',(17.8898577420822,21.1611502478916,-20.636728559038));
#90000=CARTESIAN_POINT('Ctrl Pts',(17.6564348815259,21.0350347338997,-20.6222691877976));
#90001=CARTESIAN_POINT('Ctrl Pts',(17.5874485616865,20.9924788914488,-20.6178175353737));
#90002=CARTESIAN_POINT('Ctrl Pts',(17.4913574536307,20.925305470127,-20.6111127793929));
#90003=CARTESIAN_POINT('Ctrl Pts',(17.4621801061937,20.9037721482331,-20.6090040747575));
#90004=CARTESIAN_POINT('Ctrl Pts',(17.4276696923469,20.8769069835119,-20.6064014686361));
#90005=CARTESIAN_POINT('Ctrl Pts',(17.4217917985262,20.8722810065139,-20.6059542820975));
#90006=CARTESIAN_POINT('Ctrl Pts',(17.4126815188217,20.8650325860968,-20.6052548588013));
#90007=CARTESIAN_POINT('Ctrl Pts',(17.4094320761689,20.8624315423432,-20.6050041269599));
#90008=CARTESIAN_POINT('Ctrl Pts',(17.4034133432647,20.8575846051757,-20.6045373186838));
#90009=CARTESIAN_POINT('Ctrl Pts',(17.4006420485626,20.8553412923782,-20.6043214269298));
#90010=CARTESIAN_POINT('Ctrl Pts',(17.3943809880378,20.8502468423371,-20.6038315177572));
#90011=CARTESIAN_POINT('Ctrl Pts',(17.3908946687434,20.8473915716002,-20.6035572042259));
#90012=CARTESIAN_POINT('Ctrl Pts',(17.3806055030626,20.838909786348,-20.6027431842953));
#90013=CARTESIAN_POINT('Ctrl Pts',(17.3738288038391,20.8332519063736,-20.6022012779455));
#90014=CARTESIAN_POINT('Ctrl Pts',(17.324210047106,20.7912956402657,-20.5981920259182));
#90015=CARTESIAN_POINT('Ctrl Pts',(17.282795608028,20.7533510133226,-20.5946171897731));
#90016=CARTESIAN_POINT('Ctrl Pts',(17.1985928197579,20.6698066685642,-20.5869375052346));
#90017=CARTESIAN_POINT('Ctrl Pts',(17.1562146579564,20.6238640788818,-20.5828222650344));
#90018=CARTESIAN_POINT('Ctrl Pts',(17.0452480462374,20.4923357600657,-20.571455376874));
#90019=CARTESIAN_POINT('Ctrl Pts',(16.9811726613987,20.4031846634318,-20.5642057676579));
#90020=CARTESIAN_POINT('Ctrl Pts',(16.8955510673252,20.2621239937673,-20.5535967724632));
#90021=CARTESIAN_POINT('Ctrl Pts',(16.8686817505602,20.2136688334086,-20.5500891281262));
#90022=CARTESIAN_POINT('Ctrl Pts',(16.8282391532386,20.1334695321404,-20.5445055521425));
#90023=CARTESIAN_POINT('Ctrl Pts',(16.8134880194395,20.102352003432,-20.5423907307492));
#90024=CARTESIAN_POINT('Ctrl Pts',(16.7951057146868,20.0609971092059,-20.5396455464173));
#90025=CARTESIAN_POINT('Ctrl Pts',(16.7907854904367,20.0510735157795,-20.5389916564798));
#90026=CARTESIAN_POINT('Ctrl Pts',(16.7838354325762,20.0347686479469,-20.537925086868));
#90027=CARTESIAN_POINT('Ctrl Pts',(16.7811604049575,20.0284069630021,-20.5375108717434));
#90028=CARTESIAN_POINT('Ctrl Pts',(16.7760434385899,20.0160694224975,-20.5367112474208));
#90029=CARTESIAN_POINT('Ctrl Pts',(16.7735976345372,20.0100952623573,-20.5363257105257));
#90030=CARTESIAN_POINT('Ctrl Pts',(16.768014752315,19.996278518032,-20.5354378438087));
#90031=CARTESIAN_POINT('Ctrl Pts',(16.7648971948507,19.9884281258775,-20.5349361774479));
#90032=CARTESIAN_POINT('Ctrl Pts',(16.7566421279442,19.9672726087486,-20.5335916499447));
#90033=CARTESIAN_POINT('Ctrl Pts',(16.7515918945119,19.9539337326075,-20.532751715932));
#90034=CARTESIAN_POINT('Ctrl Pts',(16.6965077126275,19.8038811152991,-20.5233872012149));
#90035=CARTESIAN_POINT('Ctrl Pts',(16.6605663579823,19.6624018962055,-20.5153746946421));
#90036=CARTESIAN_POINT('Ctrl Pts',(16.6244283768288,19.4161126844961,-20.5018389983019));
#90037=CARTESIAN_POINT('Ctrl Pts',(16.6169334233411,19.3129338000966,-20.4962758002309));
#90038=CARTESIAN_POINT('Ctrl Pts',(16.6170394068523,19.1495719686811,-20.487137402816));
#90039=CARTESIAN_POINT('Ctrl Pts',(16.6196337803189,19.0895518828876,-20.4837076735602));
#90040=CARTESIAN_POINT('Ctrl Pts',(16.6255428349016,19.0207954004558,-20.4796144316925));
#90041=CARTESIAN_POINT('Ctrl Pts',(16.6263673827784,19.0118664991852,-20.4790796684169));
#90042=CARTESIAN_POINT('Ctrl Pts',(16.6276944057823,18.998429261409,-20.4782697071146));
#90043=CARTESIAN_POINT('Ctrl Pts',(16.6281546997847,18.9939167306783,-20.4779968214312));
#90044=CARTESIAN_POINT('Ctrl Pts',(16.629002949118,18.9858574997488,-20.4775078245677));
#90045=CARTESIAN_POINT('Ctrl Pts',(16.6293853710041,18.9823102695823,-20.4772920272819));
#90046=CARTESIAN_POINT('Ctrl Pts',(16.6302310228264,18.9746480637434,-20.4768246526068));
#90047=CARTESIAN_POINT('Ctrl Pts',(16.6306973530316,18.9705335331746,-20.4765729082141));
#90048=CARTESIAN_POINT('Ctrl Pts',(16.6320285817631,18.9590880140098,-20.475870533521));
#90049=CARTESIAN_POINT('Ctrl Pts',(16.632919747666,18.9517602242514,-20.4754184636422));
#90050=CARTESIAN_POINT('Ctrl Pts',(16.6382144753014,18.9100449752937,-20.4728319180673));
#90051=CARTESIAN_POINT('Ctrl Pts',(16.6434236289392,18.8757672336488,-20.470656115383));
#90052=CARTESIAN_POINT('Ctrl Pts',(16.662592792622,18.7675851043797,-20.4636610256852));
#90053=CARTESIAN_POINT('Ctrl Pts',(16.6796496235097,18.6942916022204,-20.4587324116113));
#90054=CARTESIAN_POINT('Ctrl Pts',(16.7139659304942,18.5758064391525,-20.4505956078634));
#90055=CARTESIAN_POINT('Ctrl Pts',(16.7289275855916,18.5300554242867,-20.4474103353874));
#90056=CARTESIAN_POINT('Ctrl Pts',(16.7454193207648,18.4848898966601,-20.4442392307736));
#90057=CARTESIAN_POINT('Origin',(18.734,19.211,0.));
#90058=CARTESIAN_POINT('',(16.7454194502465,18.4848895420517,-19.6425235887674));
#90059=CARTESIAN_POINT('',(16.7452305124652,18.4848205810513,-19.866484321603));
#90060=CARTESIAN_POINT('',(16.7454194503191,18.4848895418526,0.));
#90061=CARTESIAN_POINT('',(16.6200797422209,19.2118282580408,-19.9109991802722));
#90062=CARTESIAN_POINT('Ctrl Pts',(16.7452305124652,18.4848205810513,-19.866484321603));
#90063=CARTESIAN_POINT('Ctrl Pts',(16.6631151030873,18.7170153086961,-19.8813041213945));
#90064=CARTESIAN_POINT('Ctrl Pts',(16.6210474027165,18.9645594739241,-19.896123921186));
#90065=CARTESIAN_POINT('Ctrl Pts',(16.620175975625,19.2118314138067,-19.9109437209775));
#90066=CARTESIAN_POINT('Ctrl Pts',(16.617000124922,19.2117272686677,-19.9127739632071));
#90067=CARTESIAN_POINT('Ctrl Pts',(16.6170670033201,19.4064030010461,-19.9239833213257));
#90068=CARTESIAN_POINT('Ctrl Pts',(16.6439835663,19.6001371164809,-19.9342646372126));
#90069=CARTESIAN_POINT('Ctrl Pts',(16.7140733651364,19.8478011973305,-19.948410553006));
#90070=CARTESIAN_POINT('Ctrl Pts',(16.7338151510888,19.9073323898861,-19.9519022938411));
#90071=CARTESIAN_POINT('Ctrl Pts',(16.767193688988,19.9947844752322,-19.9572865043126));
#90072=CARTESIAN_POINT('Ctrl Pts',(16.7788510569389,20.0234269518889,-19.9590922720175));
#90073=CARTESIAN_POINT('Ctrl Pts',(16.7939618108709,20.0583438699617,-19.9613581576324));
#90074=CARTESIAN_POINT('Ctrl Pts',(16.7968258155017,20.0648711758011,-19.9617845528516));
#90075=CARTESIAN_POINT('Ctrl Pts',(16.8013829439054,20.075116313182,-19.9624584414996));
#90076=CARTESIAN_POINT('Ctrl Pts',(16.8030539888956,20.0788439893012,-19.9627046029928));
#90077=CARTESIAN_POINT('Ctrl Pts',(16.8062079245867,20.0858254110863,-19.9631674899564));
#90078=CARTESIAN_POINT('Ctrl Pts',(16.8076882729767,20.0890802443747,-19.9633840592415));
#90079=CARTESIAN_POINT('Ctrl Pts',(16.8111000205985,20.0965314841062,-19.9638815930443));
#90080=CARTESIAN_POINT('Ctrl Pts',(16.8130369086226,20.1007253175883,-19.9641628924463));
#90081=CARTESIAN_POINT('Ctrl Pts',(16.8190812888894,20.1137011271452,-19.9650370990681));
#90082=CARTESIAN_POINT('Ctrl Pts',(16.823235326096,20.1224611060637,-19.9656327721567));
#90083=CARTESIAN_POINT('Ctrl Pts',(16.8705050515305,20.2203994966495,-19.9723517880548));
#90084=CARTESIAN_POINT('Ctrl Pts',(16.9197639317907,20.3064650150461,-19.9788045467882));
#90085=CARTESIAN_POINT('Ctrl Pts',(17.0685545516379,20.5287045103512,-19.9964228353183));
#90086=CARTESIAN_POINT('Ctrl Pts',(17.1786346335275,20.6569976269522,-20.0076111765957));
#90087=CARTESIAN_POINT('Ctrl Pts',(17.3256315799805,20.7918700503244,-20.0201380776319));
#90088=CARTESIAN_POINT('Ctrl Pts',(17.3489534005475,20.8123424983284,-20.0220665886807));
#90089=CARTESIAN_POINT('Ctrl Pts',(17.384311874298,20.8420303948361,-20.024904952664));
#90090=CARTESIAN_POINT('Ctrl Pts',(17.3960102342132,20.8516406038085,-20.0258306231042));
#90091=CARTESIAN_POINT('Ctrl Pts',(17.4149104263543,20.8668305033765,-20.0273050947322));
#90092=CARTESIAN_POINT('Ctrl Pts',(17.4220467681044,20.872490499702,-20.0278571078492));
#90093=CARTESIAN_POINT('Ctrl Pts',(17.4357273373919,20.8831977719531,-20.0289064532558));
#90094=CARTESIAN_POINT('Ctrl Pts',(17.4422650096485,20.8882531152831,-20.0294041017591));
#90095=CARTESIAN_POINT('Ctrl Pts',(17.4537923339595,20.8970593980031,-20.0302749615039));
#90096=CARTESIAN_POINT('Ctrl Pts',(17.4587692532811,20.900826767956,-20.0306488191648));
#90097=CARTESIAN_POINT('Ctrl Pts',(17.4686248253976,20.9082187852628,-20.0313849848409));
#90098=CARTESIAN_POINT('Ctrl Pts',(17.4735025664652,20.9118445428041,-20.0317473341812));
#90099=CARTESIAN_POINT('Ctrl Pts',(17.4852053358776,20.9204655358477,-20.0326119736801));
#90100=CARTESIAN_POINT('Ctrl Pts',(17.4920448515565,20.9254410003849,-20.033113493206));
#90101=CARTESIAN_POINT('Ctrl Pts',(17.5168619450707,20.943267964101,-20.0349197417771));
#90102=CARTESIAN_POINT('Ctrl Pts',(17.5350110552213,20.9558790527527,-20.036215244557));
#90103=CARTESIAN_POINT('Ctrl Pts',(17.7074238415235,21.0717212220229,-20.0482960856431));
#90104=CARTESIAN_POINT('Ctrl Pts',(17.8744321224907,21.1545254444176,-20.0582244906873));
#90105=CARTESIAN_POINT('Ctrl Pts',(18.1259430444054,21.2403783098153,-20.0727122644604));
#90106=CARTESIAN_POINT('Ctrl Pts',(18.2031781733303,21.261935339801,-20.0771188428785));
#90107=CARTESIAN_POINT('Ctrl Pts',(18.3166359031823,21.2867635031169,-20.0837623330807));
#90108=CARTESIAN_POINT('Ctrl Pts',(18.352018135063,21.2935648649068,-20.0858578674268));
#90109=CARTESIAN_POINT('Ctrl Pts',(18.3949195811649,21.3006816052478,-20.0884458673372));
#90110=CARTESIAN_POINT('Ctrl Pts',(18.4022912553874,21.301864425717,-20.0888922292708));
#90111=CARTESIAN_POINT('Ctrl Pts',(18.4137790899883,21.3036454234865,-20.0895906433832));
#90112=CARTESIAN_POINT('Ctrl Pts',(18.4178911013325,21.3042705183868,-20.0898411977216));
#90113=CARTESIAN_POINT('Ctrl Pts',(18.4255318938312,21.3054090200908,-20.0903078539977));
#90114=CARTESIAN_POINT('Ctrl Pts',(18.4290601396448,21.3059256304036,-20.0905237723762));
#90115=CARTESIAN_POINT('Ctrl Pts',(18.4370543996723,21.3070755369671,-20.0910139727954));
#90116=CARTESIAN_POINT('Ctrl Pts',(18.4415211202765,21.3077034721845,-20.0912885524036));
#90117=CARTESIAN_POINT('Ctrl Pts',(18.4530597186375,21.3092879890831,-20.0919995631071));
#90118=CARTESIAN_POINT('Ctrl Pts',(18.4601344213738,21.310223086848,-20.09243716118));
#90119=CARTESIAN_POINT('Ctrl Pts',(18.5036195860804,21.3157471699273,-20.0951364752464));
#90120=CARTESIAN_POINT('Ctrl Pts',(18.5401372204707,21.3194242060631,-20.0974444600204));
#90121=CARTESIAN_POINT('Ctrl Pts',(18.7466315537019,21.3348070585388,-20.110659309168));
#90122=CARTESIAN_POINT('Ctrl Pts',(18.917438746667,21.3269086167166,-20.1221549647551));
#90123=CARTESIAN_POINT('Ctrl Pts',(19.1796055634226,21.2827721816778,-20.1394327629003));
#90124=CARTESIAN_POINT('Ctrl Pts',(19.2725841369815,21.260569633114,-20.1454989500872));
#90125=CARTESIAN_POINT('Ctrl Pts',(19.3841906711131,21.2257950636535,-20.152679591087));
#90126=CARTESIAN_POINT('Ctrl Pts',(19.4045268847032,21.2191187233347,-20.1539841509957));
#90127=CARTESIAN_POINT('Ctrl Pts',(19.4332773989738,21.2091945173494,-20.155823583054));
#90128=CARTESIAN_POINT('Ctrl Pts',(19.4417770754778,21.206199695578,-20.1563667729496));
#90129=CARTESIAN_POINT('Ctrl Pts',(19.4563992918996,21.2009424266203,-20.1573002550792));
#90130=CARTESIAN_POINT('Ctrl Pts',(19.4625309177163,21.1987057884941,-20.1576913988416));
#90131=CARTESIAN_POINT('Ctrl Pts',(19.474245895529,21.194371016256,-20.1584381742853));
#90132=CARTESIAN_POINT('Ctrl Pts',(19.4798309067873,21.1922775761044,-20.1587939581181));
#90133=CARTESIAN_POINT('Ctrl Pts',(19.4943189797994,21.1867770420022,-20.1597163275077));
#90134=CARTESIAN_POINT('Ctrl Pts',(19.5032080723402,21.1833333432032,-20.1602816822379));
#90135=CARTESIAN_POINT('Ctrl Pts',(19.5333788628564,21.1714099659397,-20.1621989074506));
#90136=CARTESIAN_POINT('Ctrl Pts',(19.5545465204449,21.162644759941,-20.1635411669092));
#90137=CARTESIAN_POINT('Ctrl Pts',(19.7375871778113,21.083345785542,-20.1751335932724));
#90138=CARTESIAN_POINT('Ctrl Pts',(19.8901866707694,20.9931630098304,-20.1846219518578));
#90139=CARTESIAN_POINT('Ctrl Pts',(20.098028332902,20.8322815023627,-20.1989254521405));
#90140=CARTESIAN_POINT('Ctrl Pts',(20.1629330412029,20.7753768777675,-20.2036492252431));
#90141=CARTESIAN_POINT('Ctrl Pts',(20.2509094507185,20.6881901505228,-20.2107223713131));
#90142=CARTESIAN_POINT('Ctrl Pts',(20.2769247819386,20.6609957745515,-20.2129085161486));
#90143=CARTESIAN_POINT('Ctrl Pts',(20.3072787891831,20.6275239197596,-20.215596997621));
#90144=CARTESIAN_POINT('Ctrl Pts',(20.3123276497528,20.621896165514,-20.2160489478182));
#90145=CARTESIAN_POINT('Ctrl Pts',(20.3201207309801,20.6131153655055,-20.2167542186257));
#90146=CARTESIAN_POINT('Ctrl Pts',(20.3228860002234,20.6099809680736,-20.2170059934516));
#90147=CARTESIAN_POINT('Ctrl Pts',(20.327991831889,20.6041589075598,-20.2174737425594));
#90148=CARTESIAN_POINT('Ctrl Pts',(20.3303348968439,20.6014735158847,-20.2176895258141));
#90149=CARTESIAN_POINT('Ctrl Pts',(20.3356100772121,20.5953967131529,-20.2181779024908));
#90150=CARTESIAN_POINT('Ctrl Pts',(20.3385381904178,20.5920019165271,-20.2184507840204));
#90151=CARTESIAN_POINT('Ctrl Pts',(20.3471299313312,20.5819766100911,-20.2192567223996));
#90152=CARTESIAN_POINT('Ctrl Pts',(20.3527633196,20.5753204718402,-20.2197919160065));
#90153=CARTESIAN_POINT('Ctrl Pts',(20.3925706226343,20.527692464828,-20.2236210423224));
#90154=CARTESIAN_POINT('Ctrl Pts',(20.4252231437164,20.4854798149951,-20.2270120692406));
#90155=CARTESIAN_POINT('Ctrl Pts',(20.4665329483751,20.4276888084987,-20.2316031721895));
#90156=CARTESIAN_POINT('Ctrl Pts',(20.4766412820537,20.4131661330435,-20.2327528101188));
#90157=CARTESIAN_POINT('Ctrl Pts',(20.5137261870369,20.3584354181624,-20.2370658061026));
#90158=CARTESIAN_POINT('Ctrl Pts',(20.5395023995542,20.3174330925795,-20.2402577089861));
#90159=CARTESIAN_POINT('Ctrl Pts',(20.618854998902,20.1810387131874,-20.250681431172));
#90160=CARTESIAN_POINT('Ctrl Pts',(20.6664544649947,20.0823648366458,-20.2579141975047));
#90161=CARTESIAN_POINT('Ctrl Pts',(20.7262436204897,19.9291159278624,-20.2684877867674));
#90162=CARTESIAN_POINT('Ctrl Pts',(20.7442602346272,19.8770178221181,-20.2719769890089));
#90163=CARTESIAN_POINT('Ctrl Pts',(20.7701619401027,19.7914397319328,-20.2775346424689));
#90164=CARTESIAN_POINT('Ctrl Pts',(20.7793002306,19.7583690818511,-20.2796415347935));
#90165=CARTESIAN_POINT('Ctrl Pts',(20.7902558947884,19.7146045233436,-20.2823780853767));
#90166=CARTESIAN_POINT('Ctrl Pts',(20.7928002866236,19.7040995917341,-20.283031085991));
#90167=CARTESIAN_POINT('Ctrl Pts',(20.7968365513889,19.6868591636119,-20.2840965764876));
#90168=CARTESIAN_POINT('Ctrl Pts',(20.7983761289854,19.6801351416883,-20.2845105958338));
#90169=CARTESIAN_POINT('Ctrl Pts',(20.8012931104002,19.6671029310108,-20.2853100987148));
#90170=CARTESIAN_POINT('Ctrl Pts',(20.8026745717411,19.6607957376877,-20.2856957086015));
#90171=CARTESIAN_POINT('Ctrl Pts',(20.8057982552624,19.6462154258846,-20.2865841097924));
#90172=CARTESIAN_POINT('Ctrl Pts',(20.8075198239698,19.6379379582605,-20.2870862350647));
#90173=CARTESIAN_POINT('Ctrl Pts',(20.8120175823714,19.6156431907515,-20.2884328051846));
#90174=CARTESIAN_POINT('Ctrl Pts',(20.814701545353,19.601607576144,-20.2892743087983));
#90175=CARTESIAN_POINT('Ctrl Pts',(20.8380201751499,19.472596965349,-20.2969546458627));
#90176=CARTESIAN_POINT('Ctrl Pts',(20.8492493029019,19.3561189760174,-20.3034769374647));
#90177=CARTESIAN_POINT('Ctrl Pts',(20.8529854148806,19.0766185722943,-20.3187795159421));
#90178=CARTESIAN_POINT('Ctrl Pts',(20.8364003228626,18.9142532946038,-20.3273768859465));
#90179=CARTESIAN_POINT('Ctrl Pts',(20.7943873034294,18.7236051013331,-20.338585518038));
#90180=CARTESIAN_POINT('Ctrl Pts',(20.7866460999621,18.6919688322643,-20.3404849054904));
#90181=CARTESIAN_POINT('Ctrl Pts',(20.7762953124876,18.6535313231779,-20.3428550183296));
#90182=CARTESIAN_POINT('Ctrl Pts',(20.7743759484222,18.646546764826,-20.3432882379055));
#90183=CARTESIAN_POINT('Ctrl Pts',(20.7713112837595,18.6356143645867,-20.343970510917));
#90184=CARTESIAN_POINT('Ctrl Pts',(20.7701902442007,18.6316596983337,-20.3442181766205));
#90185=CARTESIAN_POINT('Ctrl Pts',(20.7680735885213,18.6242748565839,-20.3446823157286));
#90186=CARTESIAN_POINT('Ctrl Pts',(20.7670808067098,18.6208439272789,-20.3448986234359));
#90187=CARTESIAN_POINT('Ctrl Pts',(20.7647951422541,18.6130191747389,-20.3453934740329));
#90188=CARTESIAN_POINT('Ctrl Pts',(20.7634966847379,18.6086270400241,-20.3456723383312));
#90189=CARTESIAN_POINT('Ctrl Pts',(20.7594631138016,18.5951442572704,-20.3465316864651));
#90190=CARTESIAN_POINT('Ctrl Pts',(20.756681140914,18.5860679111297,-20.3471148050523));
#90191=CARTESIAN_POINT('Ctrl Pts',(20.7312131755112,18.5049290373252,-20.3523672096824));
#90192=CARTESIAN_POINT('Ctrl Pts',(20.7047480677554,18.4341176349763,-20.3572297750416));
#90193=CARTESIAN_POINT('Ctrl Pts',(20.6204437741514,18.2407673307749,-20.3710232150381));
#90194=CARTESIAN_POINT('Ctrl Pts',(20.5545411181801,18.1221220173689,-20.3800734118708));
#90195=CARTESIAN_POINT('Ctrl Pts',(20.4267690694175,17.9365166446469,-20.3946763522883));
#90196=CARTESIAN_POINT('Ctrl Pts',(20.3711079576764,17.8657654185015,-20.4003747605024));
#90197=CARTESIAN_POINT('Ctrl Pts',(20.2972795996307,17.7833180987809,-20.4071682347154));
#90198=CARTESIAN_POINT('Ctrl Pts',(20.2832245288497,17.7680786144507,-20.4084312197239));
#90199=CARTESIAN_POINT('Ctrl Pts',(20.262820376999,17.7465969108227,-20.4102226404648));
#90200=CARTESIAN_POINT('Ctrl Pts',(20.2566525961896,17.7401848424043,-20.4107588149748));
#90201=CARTESIAN_POINT('Ctrl Pts',(20.2459047273481,17.7291513489926,-20.4116840366499));
#90202=CARTESIAN_POINT('Ctrl Pts',(20.2413434535983,17.7245118421491,-20.4120738957558));
#90203=CARTESIAN_POINT('Ctrl Pts',(20.232542415171,17.715642016393,-20.4128208285973));
#90204=CARTESIAN_POINT('Ctrl Pts',(20.2283059510638,17.7114085239793,-20.4131780419467));
#90205=CARTESIAN_POINT('Ctrl Pts',(20.2171837811252,17.7003880892693,-20.4141098265386));
#90206=CARTESIAN_POINT('Ctrl Pts',(20.2102693971544,17.6936301883947,-20.4146831158009));
#90207=CARTESIAN_POINT('Ctrl Pts',(20.1862277696811,17.670452552023,-20.4166562195719));
#90208=CARTESIAN_POINT('Ctrl Pts',(20.1688705619979,17.6542731544564,-20.4180456362898));
#90209=CARTESIAN_POINT('Ctrl Pts',(20.0307900511407,17.5298343845559,-20.4288389213426));
#90210=CARTESIAN_POINT('Ctrl Pts',(19.898262515005,17.4354769657898,-20.4376172873601));
#90211=CARTESIAN_POINT('Ctrl Pts',(19.6420314168533,17.2941848320124,-20.4535133211676));
#90212=CARTESIAN_POINT('Ctrl Pts',(19.5222534792738,17.2419017260531,-20.4606065192551));
#90213=CARTESIAN_POINT('Ctrl Pts',(19.3871571164304,17.1972432588567,-20.4690032816716));
#90214=CARTESIAN_POINT('Ctrl Pts',(19.3758346180798,17.1936059533017,-20.4697100255689));
#90215=CARTESIAN_POINT('Ctrl Pts',(19.3596901894346,17.1885692874668,-20.4707228105304));
#90216=CARTESIAN_POINT('Ctrl Pts',(19.3548927620591,17.1870913120911,-20.4710243987553));
#90217=CARTESIAN_POINT('Ctrl Pts',(19.3466142814134,17.1845731096321,-20.4715459830214));
#90218=CARTESIAN_POINT('Ctrl Pts',(19.3431356872957,17.1835247438966,-20.4717655043885));
#90219=CARTESIAN_POINT('Ctrl Pts',(19.3363840983526,17.1815089193617,-20.472192283586));
#90220=CARTESIAN_POINT('Ctrl Pts',(19.3331114559672,17.180540418702,-20.4723994731696));
#90221=CARTESIAN_POINT('Ctrl Pts',(19.3242722228052,17.1779477803213,-20.4729599180046));
#90222=CARTESIAN_POINT('Ctrl Pts',(19.3187013255415,17.1763386072745,-20.4733140308232));
#90223=CARTESIAN_POINT('Ctrl Pts',(19.2979808492575,17.1704455498023,-20.4746342580403));
#90224=CARTESIAN_POINT('Ctrl Pts',(19.2827906697476,17.1663079376682,-20.4756083278444));
#90225=CARTESIAN_POINT('Ctrl Pts',(19.1401117360924,17.1291484034575,-20.484806486577));
#90226=CARTESIAN_POINT('Ctrl Pts',(19.0098595716459,17.1079241109576,-20.4935492165282));
#90227=CARTESIAN_POINT('Ctrl Pts',(18.7196001202769,17.0880664028084,-20.5127673929404));
#90228=CARTESIAN_POINT('Ctrl Pts',(18.5599586860911,17.0951592199509,-20.5231357200905));
#90229=CARTESIAN_POINT('Ctrl Pts',(18.3815824374086,17.1234311449658,-20.5342280935254));
#90230=CARTESIAN_POINT('Ctrl Pts',(18.3606150748576,17.1270792691412,-20.5355251291975));
#90231=CARTESIAN_POINT('Ctrl Pts',(18.3308716521736,17.1327176853398,-20.5373559034078));
#90232=CARTESIAN_POINT('Ctrl Pts',(18.3220482928543,17.134448618712,-20.5378978528596));
#90233=CARTESIAN_POINT('Ctrl Pts',(18.3068429680297,17.1375322709397,-20.5388298878122));
#90234=CARTESIAN_POINT('Ctrl Pts',(18.3004557869053,17.1388583614563,-20.5392208176929));
#90235=CARTESIAN_POINT('Ctrl Pts',(18.2882360530744,17.1414543655766,-20.5399676506761));
#90236=CARTESIAN_POINT('Ctrl Pts',(18.2824025517059,17.1427194641061,-20.5403237036971));
#90237=CARTESIAN_POINT('Ctrl Pts',(18.2672432067404,17.1460742308842,-20.5412477787271));
#90238=CARTESIAN_POINT('Ctrl Pts',(18.257925957516,17.1482024222824,-20.5418145608792));
#90239=CARTESIAN_POINT('Ctrl Pts',(18.2261824781334,17.1556796120282,-20.5437418037932));
#90240=CARTESIAN_POINT('Ctrl Pts',(18.2038288681629,17.1613319378218,-20.5450925151864));
#90241=CARTESIAN_POINT('Ctrl Pts',(18.013003440215,17.2129148153442,-20.556578359049));
#90242=CARTESIAN_POINT('Ctrl Pts',(17.8507219827634,17.2791596527801,-20.5659712393592));
#90243=CARTESIAN_POINT('Ctrl Pts',(17.6219937525634,17.4074460802779,-20.5802384872169));
#90244=CARTESIAN_POINT('Ctrl Pts',(17.5483211304217,17.4550023282368,-20.5850329287597));
#90245=CARTESIAN_POINT('Ctrl Pts',(17.4472443094895,17.5295152340532,-20.5922013604299));
#90246=CARTESIAN_POINT('Ctrl Pts',(17.4172901011136,17.552866753355,-20.5944070627951));
#90247=CARTESIAN_POINT('Ctrl Pts',(17.382131208064,17.5818292801119,-20.5971172261748));
#90248=CARTESIAN_POINT('Ctrl Pts',(17.3763062272557,17.5866804253275,-20.5975703516762));
#90249=CARTESIAN_POINT('Ctrl Pts',(17.3673067049478,17.5942576132068,-20.5982770668746));
#90250=CARTESIAN_POINT('Ctrl Pts',(17.3641139118947,17.5969620162727,-20.5985291006687));
#90251=CARTESIAN_POINT('Ctrl Pts',(17.35821696782,17.6019870273684,-20.5989970721733));
#90252=CARTESIAN_POINT('Ctrl Pts',(17.3555106504383,17.6043050039598,-20.599212817212));
#90253=CARTESIAN_POINT('Ctrl Pts',(17.3494172446107,17.6095507695748,-20.5997007814425));
#90254=CARTESIAN_POINT('Ctrl Pts',(17.3460336042783,17.6124824593874,-20.5999732866671));
#90255=CARTESIAN_POINT('Ctrl Pts',(17.3361072842766,17.6211382049902,-20.6007771919632));
#90256=CARTESIAN_POINT('Ctrl Pts',(17.3295906258286,17.6268917727313,-20.6013107135226));
#90257=CARTESIAN_POINT('Ctrl Pts',(17.2837290690074,17.6678884261223,-20.605105191026));
#90258=CARTESIAN_POINT('Ctrl Pts',(17.2456831712069,17.7045501633625,-20.6084613457161));
#90259=CARTESIAN_POINT('Ctrl Pts',(17.1955083637951,17.7566569480874,-20.613134828151));
#90260=CARTESIAN_POINT('Ctrl Pts',(17.1821607821879,17.7709079069263,-20.6144037596343));
#90261=CARTESIAN_POINT('Ctrl Pts',(17.0704029012836,17.8935878039253,-20.6252363496672));
#90262=CARTESIAN_POINT('Ctrl Pts',(16.9832805131874,18.0117849697411,-20.6350415605194));
#90263=CARTESIAN_POINT('Ctrl Pts',(16.8777709759383,18.1912387444812,-20.6484905850079));
#90264=CARTESIAN_POINT('Ctrl Pts',(16.8488257062074,18.2457962822831,-20.6524166966287));
#90265=CARTESIAN_POINT('Ctrl Pts',(16.8063135236479,18.3351579117933,-20.658582697587));
#90266=CARTESIAN_POINT('Ctrl Pts',(16.7912114314477,18.3691880444925,-20.6608723594011));
#90267=CARTESIAN_POINT('Ctrl Pts',(16.7727688479727,18.4138894368113,-20.6638069323112));
#90268=CARTESIAN_POINT('Ctrl Pts',(16.7686050585361,18.4242118372078,-20.6644796217732));
#90269=CARTESIAN_POINT('Ctrl Pts',(16.7619670934183,18.4410494996135,-20.6655689840445));
#90270=CARTESIAN_POINT('Ctrl Pts',(16.7594433795558,18.4475448853054,-20.6659873210957));
#90271=CARTESIAN_POINT('Ctrl Pts',(16.7546526122558,18.4600577481487,-20.6667896098439));
#90272=CARTESIAN_POINT('Ctrl Pts',(16.7523808176238,18.4660733160689,-20.6671737171445));
#90273=CARTESIAN_POINT('Ctrl Pts',(16.7485503973944,18.4763575531617,-20.6678277065683));
#90274=CARTESIAN_POINT('Ctrl Pts',(16.7469780570343,18.480621024627,-20.6680980434942));
#90275=CARTESIAN_POINT('Ctrl Pts',(16.7454194503208,18.4848895418481,-20.6683679253911));
#90276=CARTESIAN_POINT('',(16.6170007438876,19.2127747167393,-19.6896814481124));
#90277=CARTESIAN_POINT('Ctrl Pts',(16.7454193207648,18.4848898966601,-20.4442392307736));
#90278=CARTESIAN_POINT('Ctrl Pts',(16.7951094570157,18.3488046880358,-20.4346845890896));
#90279=CARTESIAN_POINT('Ctrl Pts',(16.8586919903781,18.2180328599362,-20.4252945852796));
#90280=CARTESIAN_POINT('Ctrl Pts',(16.9464403518679,18.076640949622,-20.4150699242177));
#90281=CARTESIAN_POINT('Ctrl Pts',(16.9579092607725,18.0587666519309,-20.4137750718324));
#90282=CARTESIAN_POINT('Ctrl Pts',(16.9742421992522,18.0341352382721,-20.4119869468974));
#90283=CARTESIAN_POINT('Ctrl Pts',(16.9788797521117,18.0272301307979,-20.4114852460803));
#90284=CARTESIAN_POINT('Ctrl Pts',(16.9869555489791,18.015357419482,-20.4106218260161));
#90285=CARTESIAN_POINT('Ctrl Pts',(16.9903745565624,18.0103769082832,-20.4102593852774));
#90286=CARTESIAN_POINT('Ctrl Pts',(16.9974994301775,18.0000926407794,-20.409510446105));
#90287=CARTESIAN_POINT('Ctrl Pts',(17.0012083895321,17.9947910961785,-20.4091240706906));
#90288=CARTESIAN_POINT('Ctrl Pts',(17.0099528054985,17.9824131287256,-20.4082212224996));
#90289=CARTESIAN_POINT('Ctrl Pts',(17.015007643309,17.975350490551,-20.4077054996938));
#90290=CARTESIAN_POINT('Ctrl Pts',(17.0315678675804,17.9525107809737,-20.4060356658415));
#90291=CARTESIAN_POINT('Ctrl Pts',(17.0432483121647,17.9368614487756,-20.4048883353177));
#90292=CARTESIAN_POINT('Ctrl Pts',(17.1041456268364,17.8575842380121,-20.3990558847617));
#90293=CARTESIAN_POINT('Ctrl Pts',(17.1567462473642,17.7966336620975,-20.3945073887811));
#90294=CARTESIAN_POINT('Ctrl Pts',(17.3295172094598,17.6180973747365,-20.3807325332093));
#90295=CARTESIAN_POINT('Ctrl Pts',(17.4602838261406,17.5117206194863,-20.3718906604477));
#90296=CARTESIAN_POINT('Ctrl Pts',(17.6034502233839,17.4211541223408,-20.362377959221));
#90297=CARTESIAN_POINT('Ctrl Pts',(17.6046648859707,17.4203874614015,-20.3622972585964));
#90298=CARTESIAN_POINT('Ctrl Pts',(17.6514511910329,17.3909238013793,-20.3591890968416));
#90299=CARTESIAN_POINT('Ctrl Pts',(17.6980965354763,17.3639774611268,-20.3560999837281));
#90300=CARTESIAN_POINT('Ctrl Pts',(17.7534420070124,17.334761371595,-20.3523862289768));
#90301=CARTESIAN_POINT('Ctrl Pts',(17.7611952461297,17.3307297339948,-20.3518648965471));
#90302=CARTESIAN_POINT('Ctrl Pts',(17.7729670160884,17.3247007820764,-20.3510713909671));
#90303=CARTESIAN_POINT('Ctrl Pts',(17.7769674110774,17.3226679956657,-20.3508013931219));
#90304=CARTESIAN_POINT('Ctrl Pts',(17.78415687445,17.3190434093554,-20.3503154909686));
#90305=CARTESIAN_POINT('Ctrl Pts',(17.7873435244899,17.3174469320561,-20.3500998841084));
#90306=CARTESIAN_POINT('Ctrl Pts',(17.7942733320142,17.3139970386509,-20.3496304933057));
#90307=CARTESIAN_POINT('Ctrl Pts',(17.798017898015,17.3121466749749,-20.3493765292322));
#90308=CARTESIAN_POINT('Ctrl Pts',(17.8085434240306,17.3069842233638,-20.3486618058049));
#90309=CARTESIAN_POINT('Ctrl Pts',(17.8153365749291,17.3036973341438,-20.3481995251479));
#90310=CARTESIAN_POINT('Ctrl Pts',(17.8558881362349,17.2843432208021,-20.3454346602757));
#90311=CARTESIAN_POINT('Ctrl Pts',(17.8900475910066,17.2691373054308,-20.3430839405494));
#90312=CARTESIAN_POINT('Ctrl Pts',(18.0034021983097,17.2222338429609,-20.3352546371643));
#90313=CARTESIAN_POINT('Ctrl Pts',(18.0841091410243,17.1944177488118,-20.3296382492006));
#90314=CARTESIAN_POINT('Ctrl Pts',(18.3376594501303,17.1238357381799,-20.3122512658053));
#90315=CARTESIAN_POINT('Ctrl Pts',(18.5144187994228,17.0979100826066,-20.3005605642841));
#90316=CARTESIAN_POINT('Ctrl Pts',(18.7151581518733,17.0939610613943,-20.2882046004458));
#90317=CARTESIAN_POINT('Ctrl Pts',(18.7379611010077,17.0938809064429,-20.2868128514246));
#90318=CARTESIAN_POINT('Ctrl Pts',(18.7702757283948,17.0942894377574,-20.28485664383));
#90319=CARTESIAN_POINT('Ctrl Pts',(18.7797890394258,17.0944738600074,-20.2842827146958));
#90320=CARTESIAN_POINT('Ctrl Pts',(18.7952600142245,17.0948781353936,-20.2833524899106));
#90321=CARTESIAN_POINT('Ctrl Pts',(18.8012184839367,17.0950590245106,-20.28299497837));
#90322=CARTESIAN_POINT('Ctrl Pts',(18.8137017532411,17.0954907788277,-20.2822475252268));
#90323=CARTESIAN_POINT('Ctrl Pts',(18.8202263250073,17.0957466684382,-20.2818577450732));
#90324=CARTESIAN_POINT('Ctrl Pts',(18.8357680937032,17.0964282363634,-20.2809313404213));
#90325=CARTESIAN_POINT('Ctrl Pts',(18.8447840042838,17.0968814137556,-20.2803955832328));
#90326=CARTESIAN_POINT('Ctrl Pts',(18.8752566420369,17.0986085676984,-20.2785901924775));
#90327=CARTESIAN_POINT('Ctrl Pts',(18.8966972190901,17.1001516712112,-20.2773289930256));
#90328=CARTESIAN_POINT('Ctrl Pts',(19.0968831507863,17.1176276483302,-20.265629100803));
#90329=CARTESIAN_POINT('Ctrl Pts',(19.2729427661926,17.1558991105659,-20.2559871738058));
#90330=CARTESIAN_POINT('Ctrl Pts',(19.55563534682,17.2562304319389,-20.2396619613805));
#90331=CARTESIAN_POINT('Ctrl Pts',(19.665528929809,17.306149852173,-20.2330511530822));
#90332=CARTESIAN_POINT('Ctrl Pts',(19.7788432136098,17.3697825131858,-20.225348983304));
#90333=CARTESIAN_POINT('Ctrl Pts',(19.7870915041383,17.3744876937277,-20.224782954918));
#90334=CARTESIAN_POINT('Ctrl Pts',(19.7992711526086,17.3815445198093,-20.2239387186065));
#90335=CARTESIAN_POINT('Ctrl Pts',(19.8032271129766,17.383853765417,-20.223663182423));
#90336=CARTESIAN_POINT('Ctrl Pts',(19.8102543767232,17.3879864853511,-20.2231713033203));
#90337=CARTESIAN_POINT('Ctrl Pts',(19.8133285905668,17.3898049112292,-20.2229552893266));
#90338=CARTESIAN_POINT('Ctrl Pts',(19.8199306039365,17.3937326510743,-20.2224895818453));
#90339=CARTESIAN_POINT('Ctrl Pts',(19.8234568151281,17.3958444305393,-20.2222397327143));
#90340=CARTESIAN_POINT('Ctrl Pts',(19.8331790620241,17.4017054309922,-20.2215478438911));
#90341=CARTESIAN_POINT('Ctrl Pts',(19.8393619751074,17.4054761568096,-20.2211044324042));
#90342=CARTESIAN_POINT('Ctrl Pts',(19.873223284115,17.4263660121669,-20.2186578316101));
#90343=CARTESIAN_POINT('Ctrl Pts',(19.9005218241838,17.4440889309403,-20.2166182827177));
#90344=CARTESIAN_POINT('Ctrl Pts',(20.0617804767118,17.5541481560703,-20.2042121260728));
#90345=CARTESIAN_POINT('Ctrl Pts',(20.1851376989531,17.6610456984756,-20.1932557450537));
#90346=CARTESIAN_POINT('Ctrl Pts',(20.3739364296115,17.8671467048019,-20.1749987294241));
#90347=CARTESIAN_POINT('Ctrl Pts',(20.4455836710734,17.9596717797892,-20.1675581114734));
#90348=CARTESIAN_POINT('Ctrl Pts',(20.5170242791566,18.0696334490762,-20.1595512628849));
#90349=CARTESIAN_POINT('Ctrl Pts',(20.524687757949,18.0816946591474,-20.158683290665));
#90350=CARTESIAN_POINT('Ctrl Pts',(20.536690218276,18.1010142094309,-20.1573089875403));
#90351=CARTESIAN_POINT('Ctrl Pts',(20.5411087453653,18.1082223868808,-20.1567997285898));
#90352=CARTESIAN_POINT('Ctrl Pts',(20.548825353746,18.1209818238136,-20.1559043530417));
#90353=CARTESIAN_POINT('Ctrl Pts',(20.5521414191056,18.1265220285402,-20.1555175803213));
#90354=CARTESIAN_POINT('Ctrl Pts',(20.5589476833768,18.1380123318585,-20.1547195132047));
#90355=CARTESIAN_POINT('Ctrl Pts',(20.562434254574,18.1439644984921,-20.1543083541904));
#90356=CARTESIAN_POINT('Ctrl Pts',(20.5713091275901,18.1592866376952,-20.1532556456487));
#90357=CARTESIAN_POINT('Ctrl Pts',(20.5766549174612,18.1686811003867,-20.1526156374255));
#90358=CARTESIAN_POINT('Ctrl Pts',(20.5986660895473,18.2080612082621,-20.1499549702035));
#90359=CARTESIAN_POINT('Ctrl Pts',(20.6146738802308,18.2384097479925,-20.1479578400622));
#90360=CARTESIAN_POINT('Ctrl Pts',(20.6544542897448,18.3184861920493,-20.1428137541068));
#90361=CARTESIAN_POINT('Ctrl Pts',(20.6770357547662,18.3687777742881,-20.1397061875812));
#90362=CARTESIAN_POINT('Ctrl Pts',(20.7384920387879,18.5213208553026,-20.1305617656709));
#90363=CARTESIAN_POINT('Ctrl Pts',(20.7714353469632,18.6257618034146,-20.1246736398536));
#90364=CARTESIAN_POINT('Ctrl Pts',(20.8065061135522,18.7768346781319,-20.1162298807359));
#90365=CARTESIAN_POINT('Ctrl Pts',(20.8154023161376,18.821711831227,-20.1137289265928));
#90366=CARTESIAN_POINT('Ctrl Pts',(20.8265388066548,18.8893035146133,-20.1099303719367));
#90367=CARTESIAN_POINT('Ctrl Pts',(20.8298771683697,18.9118242497901,-20.1086594736193));
#90368=CARTESIAN_POINT('Ctrl Pts',(20.83297703449,18.9353456325496,-20.1073227477522));
#90369=CARTESIAN_POINT('Ctrl Pts',(20.8331018207595,18.9362974923838,-20.1072686373755));
#90370=CARTESIAN_POINT('Ctrl Pts',(20.8354237709073,18.9541031105657,-20.1062561377202));
#90371=CARTESIAN_POINT('Ctrl Pts',(20.8374184851179,18.9709822396471,-20.1052912359404));
#90372=CARTESIAN_POINT('Ctrl Pts',(20.8428741287167,19.0224587337404,-20.1023282493572));
#90373=CARTESIAN_POINT('Ctrl Pts',(20.8456859739245,19.0571171422363,-20.100305447186));
#90374=CARTESIAN_POINT('Ctrl Pts',(20.8480377917233,19.0988287089154,-20.0978209177924));
#90375=CARTESIAN_POINT('Ctrl Pts',(20.848397780341,19.1058324823669,-20.0974020474362));
#90376=CARTESIAN_POINT('Ctrl Pts',(20.8489303620409,19.1173059700972,-20.0967128982812));
#90377=CARTESIAN_POINT('Ctrl Pts',(20.8491236036519,19.121774734787,-20.096443748811));
#90378=CARTESIAN_POINT('Ctrl Pts',(20.8494453400723,19.1298044927019,-20.0959587495865));
#90379=CARTESIAN_POINT('Ctrl Pts',(20.8495790078724,19.1333652243882,-20.0957431924547));
#90380=CARTESIAN_POINT('Ctrl Pts',(20.8498502177277,19.141111561245,-20.0952731770432));
#90381=CARTESIAN_POINT('Ctrl Pts',(20.8499843282821,19.1452971880862,-20.0950185346279));
#90382=CARTESIAN_POINT('Ctrl Pts',(20.8503267812669,19.1570771596271,-20.0943000228492));
#90383=CARTESIAN_POINT('Ctrl Pts',(20.8505066611533,19.1646721779322,-20.0938346067005));
#90384=CARTESIAN_POINT('Ctrl Pts',(20.8513458920726,19.210534729721,-20.0910118009918));
#90385=CARTESIAN_POINT('Ctrl Pts',(20.8510082092333,19.2488108662269,-20.0886039480136));
#90386=CARTESIAN_POINT('Ctrl Pts',(20.8464434638979,19.3757909155159,-20.080488521367));
#90387=CARTESIAN_POINT('Ctrl Pts',(20.837673941922,19.4642339218762,-20.0746327658124));
#90388=CARTESIAN_POINT('Ctrl Pts',(20.7955385104864,19.7225135177095,-20.0573405881421));
#90389=CARTESIAN_POINT('Ctrl Pts',(20.7468892543734,19.8891492761447,-20.0459988291737));
#90390=CARTESIAN_POINT('Ctrl Pts',(20.6693363086393,20.069311835175,-20.0339236085031));
#90391=CARTESIAN_POINT('Ctrl Pts',(20.659826333289,20.0904423431364,-20.0325090175927));
#90392=CARTESIAN_POINT('Ctrl Pts',(20.6458983529489,20.1200794130089,-20.0305266084104));
#90393=CARTESIAN_POINT('Ctrl Pts',(20.6417668286636,20.1287180521974,-20.0299489719761));
#90394=CARTESIAN_POINT('Ctrl Pts',(20.6349635673037,20.1426985469259,-20.0290143826255));
#90395=CARTESIAN_POINT('Ctrl Pts',(20.6323276219431,20.1480575795881,-20.0286561910765));
#90396=CARTESIAN_POINT('Ctrl Pts',(20.6267666007581,20.1592436946251,-20.0279086139702));
#90397=CARTESIAN_POINT('Ctrl Pts',(20.6238372083006,20.1650685703505,-20.0275193841726));
#90398=CARTESIAN_POINT('Ctrl Pts',(20.6168118450126,20.1788786568011,-20.0265966400399));
#90399=CARTESIAN_POINT('Ctrl Pts',(20.6126918949556,20.1868515797068,-20.0260639746937));
#90400=CARTESIAN_POINT('Ctrl Pts',(20.5986777256448,20.2135540683878,-20.0242799973124));
#90401=CARTESIAN_POINT('Ctrl Pts',(20.5885529357114,20.2321616606394,-20.0230368453451));
#90402=CARTESIAN_POINT('Ctrl Pts',(20.5321660056872,20.3321852333781,-20.0163493070367));
#90403=CARTESIAN_POINT('Ctrl Pts',(20.4808176932904,20.4106200244604,-20.011093074299));
#90404=CARTESIAN_POINT('Ctrl Pts',(20.3294248105633,20.611435744796,-19.9972477043145));
#90405=CARTESIAN_POINT('Ctrl Pts',(20.2206238157918,20.7264348672007,-19.9889097799719));
#90406=CARTESIAN_POINT('Ctrl Pts',(20.085155597946,20.8408614855524,-19.9789094993389));
#90407=CARTESIAN_POINT('Ctrl Pts',(20.070072716307,20.8532483264439,-19.9778002284386));
#90408=CARTESIAN_POINT('Ctrl Pts',(20.0295089309296,20.8856327032057,-19.9748214525541));
#90409=CARTESIAN_POINT('Ctrl Pts',(20.0037377900495,20.9052561105954,-19.9729335674327));
#90410=CARTESIAN_POINT('Ctrl Pts',(19.9719831792781,20.9283041648871,-19.9705992232097));
#90411=CARTESIAN_POINT('Ctrl Pts',(19.9664186391456,20.9323019031832,-19.9701898668058));
#90412=CARTESIAN_POINT('Ctrl Pts',(19.9572299776596,20.938835926303,-19.969513239724));
#90413=CARTESIAN_POINT('Ctrl Pts',(19.9536170911705,20.9413880248592,-19.9692470299863));
#90414=CARTESIAN_POINT('Ctrl Pts',(19.9470815811581,20.9459739928504,-19.968765118753));
#90415=CARTESIAN_POINT('Ctrl Pts',(19.944161806287,20.9480118251388,-19.9685496930646));
#90416=CARTESIAN_POINT('Ctrl Pts',(19.9377636838038,20.9524533786159,-19.9680773381431));
#90417=CARTESIAN_POINT('Ctrl Pts',(19.9342833133151,20.9548540200928,-19.9678202102555));
#90418=CARTESIAN_POINT('Ctrl Pts',(19.9243754486021,20.9616444168809,-19.9670877607319));
#90419=CARTESIAN_POINT('Ctrl Pts',(19.91793098244,20.9660091189213,-19.9666107969111));
#90420=CARTESIAN_POINT('Ctrl Pts',(19.8767482323292,20.9935712756114,-19.9635600755652));
#90421=CARTESIAN_POINT('Ctrl Pts',(19.8413563079454,21.0157701634958,-19.9609261472213));
#90422=CARTESIAN_POINT('Ctrl Pts',(19.6395355693048,21.1341866667008,-19.9459377789451));
#90423=CARTESIAN_POINT('Ctrl Pts',(19.4612564030848,21.2084364265669,-19.9329169427359));
#90424=CARTESIAN_POINT('Ctrl Pts',(19.2540212365793,21.2632561548984,-19.9191612501326));
#90425=CARTESIAN_POINT('Ctrl Pts',(19.2325683661098,21.2685730961572,-19.9177514742479));
#90426=CARTESIAN_POINT('Ctrl Pts',(19.1536498796683,21.2868256808884,-19.9126185722941));
#90427=CARTESIAN_POINT('Ctrl Pts',(19.0957313323204,21.2976982998993,-19.9089552601452));
#90428=CARTESIAN_POINT('Ctrl Pts',(19.0253362304984,21.3078933032022,-19.9046242368097));
#90429=CARTESIAN_POINT('Ctrl Pts',(19.0132274407544,21.3095400568895,-19.9038835015789));
#90430=CARTESIAN_POINT('Ctrl Pts',(18.9932448755306,21.3120815960814,-19.9026679476835));
#90431=CARTESIAN_POINT('Ctrl Pts',(18.9853792503067,21.3130371676208,-19.9021912196226));
#90432=CARTESIAN_POINT('Ctrl Pts',(18.9711788303664,21.3146814879064,-19.9013336332256));
#90433=CARTESIAN_POINT('Ctrl Pts',(18.9648459699464,21.3153858343157,-19.9009522873901));
#90434=CARTESIAN_POINT('Ctrl Pts',(18.9512983059785,21.3168307258475,-19.9001388121778));
#90435=CARTESIAN_POINT('Ctrl Pts',(18.9440826675226,21.3175628104853,-19.8997069538151));
#90436=CARTESIAN_POINT('Ctrl Pts',(18.9245090377018,21.3194471418206,-19.8985391994712));
#90437=CARTESIAN_POINT('Ctrl Pts',(18.9121443229789,21.3205278271144,-19.8978055583238));
#90438=CARTESIAN_POINT('Ctrl Pts',(18.8484139041408,21.3255335756306,-19.894044088778));
#90439=CARTESIAN_POINT('Ctrl Pts',(18.7969244025949,21.3276917430525,-19.8910721249936));
#90440=CARTESIAN_POINT('Ctrl Pts',(18.5728865572419,21.3288986366361,-19.8783578230477));
#90441=CARTESIAN_POINT('Ctrl Pts',(18.4009110296881,21.3087378002402,-19.8692175386638));
#90442=CARTESIAN_POINT('Ctrl Pts',(18.1458531918414,21.2466497309787,-19.8547940556994));
#90443=CARTESIAN_POINT('Ctrl Pts',(18.059876760204,21.2198156477527,-19.8497581624898));
#90444=CARTESIAN_POINT('Ctrl Pts',(17.9668659605149,21.1841415467889,-19.8438559575789));
#90445=CARTESIAN_POINT('Ctrl Pts',(17.9578762415875,21.180622832386,-19.8432806405838));
#90446=CARTESIAN_POINT('Ctrl Pts',(17.9446283920641,21.175332642627,-19.842425181036));
#90447=CARTESIAN_POINT('Ctrl Pts',(17.940351333229,21.1736084834004,-19.8421478143613));
#90448=CARTESIAN_POINT('Ctrl Pts',(17.9327687443787,21.1705229661533,-19.8416539253669));
#90449=CARTESIAN_POINT('Ctrl Pts',(17.9294609936926,21.1691671958705,-19.8414377423418));
#90450=CARTESIAN_POINT('Ctrl Pts',(17.9223759646983,21.1662422241238,-19.8409730972151));
#90451=CARTESIAN_POINT('Ctrl Pts',(17.918599852042,21.1646704757281,-19.8407244869627));
#90452=CARTESIAN_POINT('Ctrl Pts',(17.9083668935981,21.1603763300653,-19.8400481911202));
#90453=CARTESIAN_POINT('Ctrl Pts',(17.9019190381823,21.1576328293799,-19.8396192557389));
#90454=CARTESIAN_POINT('Ctrl Pts',(17.8682577773545,21.1431124890333,-19.837365775939));
#90455=CARTESIAN_POINT('Ctrl Pts',(17.8412818606033,21.1307974848635,-19.8355111455508));
#90456=CARTESIAN_POINT('Ctrl Pts',(17.7614691595869,21.0923156645977,-19.8298961231196));
#90457=CARTESIAN_POINT('Ctrl Pts',(17.7094595091302,21.0645049725264,-19.8260668971797));
#90458=CARTESIAN_POINT('Ctrl Pts',(17.5778274998539,20.9868842380858,-19.81604072932));
#90459=CARTESIAN_POINT('Ctrl Pts',(17.5002332541628,20.9338812185698,-19.8097994804667));
#90460=CARTESIAN_POINT('Ctrl Pts',(17.3244637011971,20.7958346248445,-19.7951389992581));
#90461=CARTESIAN_POINT('Ctrl Pts',(17.2300711467867,20.7065607221792,-19.7868399698015));
#90462=CARTESIAN_POINT('Ctrl Pts',(17.1340194027413,20.5973619455243,-19.7779590533407));
#90463=CARTESIAN_POINT('Ctrl Pts',(17.1237432475517,20.5854128083935,-19.7770022097991));
#90464=CARTESIAN_POINT('Ctrl Pts',(17.1084069752401,20.5671716218917,-19.7755636315011));
#90465=CARTESIAN_POINT('Ctrl Pts',(17.1032480138184,20.5609637449033,-19.7750778495655));
#90466=CARTESIAN_POINT('Ctrl Pts',(17.0940714623327,20.5497920554364,-19.7742103486278));
#90467=CARTESIAN_POINT('Ctrl Pts',(17.0900406107421,20.544839309741,-19.7738280934817));
#90468=CARTESIAN_POINT('Ctrl Pts',(17.0815397717946,20.5342971753022,-19.7730193399167));
#90469=CARTESIAN_POINT('Ctrl Pts',(17.0770755863145,20.5287031946639,-19.7725930779458));
#90470=CARTESIAN_POINT('Ctrl Pts',(17.0652157884595,20.5136863538956,-19.7714564059599));
#90471=CARTESIAN_POINT('Ctrl Pts',(17.0578715697348,20.5042230957822,-19.7707480473508));
#90472=CARTESIAN_POINT('Ctrl Pts',(17.0226437435007,20.4580266781723,-19.7673276240952));
#90473=CARTESIAN_POINT('Ctrl Pts',(16.9958839238421,20.4204497673187,-19.7646597669655));
#90474=CARTESIAN_POINT('Ctrl Pts',(16.9201884532234,20.3064483393434,-19.7568622611088));
#90475=CARTESIAN_POINT('Ctrl Pts',(16.8749127709369,20.227718291307,-19.7518591836261));
#90476=CARTESIAN_POINT('Ctrl Pts',(16.8016346996246,20.0789268562845,-19.742813827327));
#90477=CARTESIAN_POINT('Ctrl Pts',(16.7720548873629,20.0098140435765,-19.7387593446402));
#90478=CARTESIAN_POINT('Ctrl Pts',(16.7108960476806,19.8428844124266,-19.7290395779754));
#90479=CARTESIAN_POINT('Ctrl Pts',(16.6826432394489,19.7440640634662,-19.7233423083425));
#90480=CARTESIAN_POINT('Ctrl Pts',(16.6596911820583,19.6341144339448,-19.7166879664956));
#90481=CARTESIAN_POINT('Ctrl Pts',(16.6577762606434,19.6246156095647,-19.7161105263504));
#90482=CARTESIAN_POINT('Ctrl Pts',(16.6550450438842,19.6105705463484,-19.715252503474));
#90483=CARTESIAN_POINT('Ctrl Pts',(16.6541782774247,19.6060340902309,-19.7149747206897));
#90484=CARTESIAN_POINT('Ctrl Pts',(16.6526668244177,19.5979806161788,-19.7144803727382));
#90485=CARTESIAN_POINT('Ctrl Pts',(16.6520161959579,19.594464763146,-19.7142641492217));
#90486=CARTESIAN_POINT('Ctrl Pts',(16.6506411799459,19.5869278126374,-19.7137997361241));
#90487=CARTESIAN_POINT('Ctrl Pts',(16.649919536023,19.5829063221139,-19.7135514000579));
#90488=CARTESIAN_POINT('Ctrl Pts',(16.6484624925562,19.5746492623871,-19.7130404378394));
#90489=CARTESIAN_POINT('Ctrl Pts',(16.6477283444895,19.5704134939939,-19.7127777435228));
#90490=CARTESIAN_POINT('Ctrl Pts',(16.6459030700641,19.559688277618,-19.7121111772311));
#90491=CARTESIAN_POINT('Ctrl Pts',(16.6448292996858,19.553195976245,-19.7117063806325));
#90492=CARTESIAN_POINT('Ctrl Pts',(16.6260483507081,19.4362572281377,-19.7043930651482));
#90493=CARTESIAN_POINT('Ctrl Pts',(16.6170944881852,19.3245991019815,-19.6970632334726));
#90494=CARTESIAN_POINT('Ctrl Pts',(16.6170007438876,19.2127747167393,-19.6896814481124));
#90495=CARTESIAN_POINT('Ctrl Pts',(16.6170007453285,19.2127764346725,-19.6896815615171));
#90496=CARTESIAN_POINT('Ctrl Pts',(16.6169163433609,19.1121935620679,-19.6830418547794));
#90497=CARTESIAN_POINT('Ctrl Pts',(16.6240004448591,19.011723653978,-19.6763771951571));
#90498=CARTESIAN_POINT('Ctrl Pts',(16.6507394666926,18.824217512163,-19.6641100541146));
#90499=CARTESIAN_POINT('Ctrl Pts',(16.6687967940729,18.7371705642616,-19.6584854932288));
#90500=CARTESIAN_POINT('Ctrl Pts',(16.697713687571,18.6316459983499,-19.6517701141624));
#90501=CARTESIAN_POINT('Ctrl Pts',(16.703445317346,18.6118666816241,-19.650515670969));
#90502=CARTESIAN_POINT('Ctrl Pts',(16.7120584357468,18.5836882444869,-19.6487341358836));
#90503=CARTESIAN_POINT('Ctrl Pts',(16.7147054415501,18.5752192061564,-19.6481994217554));
#90504=CARTESIAN_POINT('Ctrl Pts',(16.7193842606274,18.5605734498584,-19.6472759140045));
#90505=CARTESIAN_POINT('Ctrl Pts',(16.7213914142644,18.5543890371431,-19.6468863166421));
#90506=CARTESIAN_POINT('Ctrl Pts',(16.7253038020368,18.542520741734,-19.6461393276805));
#90507=CARTESIAN_POINT('Ctrl Pts',(16.7272047463052,18.5368355205668,-19.6457817991304));
#90508=CARTESIAN_POINT('Ctrl Pts',(16.7322440872851,18.5219743757202,-19.6448479608351));
#90509=CARTESIAN_POINT('Ctrl Pts',(16.7354214541583,18.5128117403889,-19.6442729442935));
#90510=CARTESIAN_POINT('Ctrl Pts',(16.7408847780493,18.4973999849371,-19.6433068766095));
#90511=CARTESIAN_POINT('Ctrl Pts',(16.7431373831887,18.4911393820238,-19.6429147521337));
#90512=CARTESIAN_POINT('Ctrl Pts',(16.7454194502465,18.4848895420517,-19.6425235887674));
#90513=CARTESIAN_POINT('Origin',(18.734,19.211,0.));
#90514=CARTESIAN_POINT('',(16.7454194035981,18.4848896698064,-18.845275399947));
#90515=CARTESIAN_POINT('',(16.7454194503191,18.4848895418526,-19.066324519095));
#90516=CARTESIAN_POINT('',(16.7454194503191,18.4848895418526,0.));
#90517=CARTESIAN_POINT('',(16.6180378694014,19.2091158125651,-19.1109437209775));
#90518=CARTESIAN_POINT('Ctrl Pts',(16.7454194503191,18.4848895418526,-19.066324519095));
#90519=CARTESIAN_POINT('Ctrl Pts',(16.7290739265814,18.5296546188661,-19.0692018281724));
#90520=CARTESIAN_POINT('Ctrl Pts',(16.7142587320644,18.5749225375465,-19.0720791372497));
#90521=CARTESIAN_POINT('Ctrl Pts',(16.7009992479655,18.6205790127144,-19.074956446327));
#90522=CARTESIAN_POINT('Ctrl Pts',(16.6758066766554,18.7073247712869,-19.0804232362542));
#90523=CARTESIAN_POINT('Ctrl Pts',(16.6561521069702,18.7957464915279,-19.0858900261814));
#90524=CARTESIAN_POINT('Ctrl Pts',(16.6422180861817,18.885212607637,-19.0913568161086));
#90525=CARTESIAN_POINT('Ctrl Pts',(16.6285119268907,18.9732156942664,-19.0967342082262));
#90526=CARTESIAN_POINT('Ctrl Pts',(16.6203407792442,19.0622293912807,-19.1021116003437));
#90527=CARTESIAN_POINT('Ctrl Pts',(16.6178326248363,19.1516313189224,-19.1074889924612));
#90528=CARTESIAN_POINT('Ctrl Pts',(16.6172955000016,19.1707768689146,-19.1086405686333));
#90529=CARTESIAN_POINT('Ctrl Pts',(16.6170179137274,19.1899401417913,-19.1097921448054));
#90530=CARTESIAN_POINT('Ctrl Pts',(16.6170008393112,19.2091148891275,-19.1109437209775));
#90531=CARTESIAN_POINT('Ctrl Pts',(16.6180378694014,19.2091158125651,-19.1109437209775));
#90532=CARTESIAN_POINT('Ctrl Pts',(16.6223667223562,19.7149949952687,-19.1413398983212));
#90533=CARTESIAN_POINT('Ctrl Pts',(17.0578063895244,20.9330881407267,-19.2141280112252));
#90534=CARTESIAN_POINT('Ctrl Pts',(19.0938031815268,21.6882711475644,-19.3293080596899));
#90535=CARTESIAN_POINT('Ctrl Pts',(21.0117476411797,20.249362367724,-19.4564838663713));
#90536=CARTESIAN_POINT('Ctrl Pts',(20.8400000149027,17.8578205193087,-19.5836596730528));
#90537=CARTESIAN_POINT('Ctrl Pts',(18.7361280844105,16.7077369418623,-19.7108354797341));
#90538=CARTESIAN_POINT('Ctrl Pts',(17.1750895095576,17.5576360166973,-19.8051103625842));
#90539=CARTESIAN_POINT('Ctrl Pts',(16.7978195031743,18.3361166232031,-19.8569933098738));
#90540=CARTESIAN_POINT('Ctrl Pts',(16.7452305124652,18.4848205810513,-19.866484321603));
#90541=CARTESIAN_POINT('Ctrl Pts',(16.7454194502465,18.4848895420517,-19.6425235887674));
#90542=CARTESIAN_POINT('Ctrl Pts',(16.7513354922673,18.4686874257408,-19.6415095349059));
#90543=CARTESIAN_POINT('Ctrl Pts',(16.7574495349329,18.4525576420121,-19.6405019471072));
#90544=CARTESIAN_POINT('Ctrl Pts',(16.8210985510288,18.2906410055608,-19.630401539589));
#90545=CARTESIAN_POINT('Ctrl Pts',(16.8944570177936,18.1515939492392,-19.6218931420355));
#90546=CARTESIAN_POINT('Ctrl Pts',(17.0277672172459,17.9552320220489,-19.6090034063394));
#90547=CARTESIAN_POINT('Ctrl Pts',(17.0768009080434,17.8911994892854,-19.604626137739));
#90548=CARTESIAN_POINT('Ctrl Pts',(17.1558585034803,17.7993313055239,-19.5978417486546));
#90549=CARTESIAN_POINT('Ctrl Pts',(17.1832341456381,17.7693121149191,-19.5955350803859));
#90550=CARTESIAN_POINT('Ctrl Pts',(17.2274000528777,17.7235954537048,-19.5918441208389));
#90551=CARTESIAN_POINT('Ctrl Pts',(17.2436121369262,17.7073512360309,-19.5904952799347));
#90552=CARTESIAN_POINT('Ctrl Pts',(17.2647242231728,17.6868741937084,-19.5887411943746));
#90553=CARTESIAN_POINT('Ctrl Pts',(17.2693846473904,17.6823951955441,-19.5883541338572));
#90554=CARTESIAN_POINT('Ctrl Pts',(17.2765098109158,17.6756099055338,-19.5877624579846));
#90555=CARTESIAN_POINT('Ctrl Pts',(17.2789597241795,17.6732880019862,-19.5875590320492));
#90556=CARTESIAN_POINT('Ctrl Pts',(17.2840076628687,17.6685266865125,-19.5871398876463));
#90557=CARTESIAN_POINT('Ctrl Pts',(17.2866062745757,17.6660879948744,-19.5869241170202));
#90558=CARTESIAN_POINT('Ctrl Pts',(17.2924855853297,17.6605983541618,-19.5864359426865));
#90559=CARTESIAN_POINT('Ctrl Pts',(17.2957697997764,17.6575512684896,-19.5861632519385));
#90560=CARTESIAN_POINT('Ctrl Pts',(17.305464263719,17.6486138640673,-19.5853583984496));
#90561=CARTESIAN_POINT('Ctrl Pts',(17.3119011128783,17.642752718206,-19.5848241074302));
#90562=CARTESIAN_POINT('Ctrl Pts',(17.3578525104004,17.6014266866031,-19.5810118571994));
#90563=CARTESIAN_POINT('Ctrl Pts',(17.3986495521066,17.5674227057259,-19.5776377272081));
#90564=CARTESIAN_POINT('Ctrl Pts',(17.452186768306,17.5261097408508,-19.573267983812));
#90565=CARTESIAN_POINT('Ctrl Pts',(17.4637871634084,17.5173472368749,-19.5723244435688));
#90566=CARTESIAN_POINT('Ctrl Pts',(17.5917504829377,17.42274270243,-19.5619592933419));
#90567=CARTESIAN_POINT('Ctrl Pts',(17.7165273210169,17.348917410824,-19.552272336456));
#90568=CARTESIAN_POINT('Ctrl Pts',(17.9293682558012,17.2508186041958,-19.5370858385326));
#90569=CARTESIAN_POINT('Ctrl Pts',(18.0131877941661,17.2184697766245,-19.5313990558285));
#90570=CARTESIAN_POINT('Ctrl Pts',(18.1185717919286,17.1853233382743,-19.5246178700095));
#90571=CARTESIAN_POINT('Ctrl Pts',(18.1384162424899,17.1794001740588,-19.5233562283486));
#90572=CARTESIAN_POINT('Ctrl Pts',(18.1669029171781,17.1713507692091,-19.5215663617672));
#90573=CARTESIAN_POINT('Ctrl Pts',(18.175476110062,17.1689864951104,-19.5210304164706));
#90574=CARTESIAN_POINT('Ctrl Pts',(18.1903461411556,17.1649863631273,-19.520105463878));
#90575=CARTESIAN_POINT('Ctrl Pts',(18.196636042038,17.163325392389,-19.5197156459303));
#90576=CARTESIAN_POINT('Ctrl Pts',(18.2087319605123,17.1601908021249,-19.5189687046807));
#90577=CARTESIAN_POINT('Ctrl Pts',(18.2145367632638,17.1587127817454,-19.5186114421817));
#90578=CARTESIAN_POINT('Ctrl Pts',(18.2297315446572,17.154912480575,-19.517679337098));
#90579=CARTESIAN_POINT('Ctrl Pts',(18.239131372457,17.1526298659422,-19.5171057782452));
#90580=CARTESIAN_POINT('Ctrl Pts',(18.2716674053281,17.1449647118447,-19.5151307937676));
#90581=CARTESIAN_POINT('Ctrl Pts',(18.2948788631051,17.1399070677099,-19.5137397928997));
#90582=CARTESIAN_POINT('Ctrl Pts',(18.4764690829838,17.1035298024291,-19.5029863845032));
#90583=CARTESIAN_POINT('Ctrl Pts',(18.6378759286409,17.0900285354248,-19.494243235366));
#90584=CARTESIAN_POINT('Ctrl Pts',(18.9302246812665,17.0990454625842,-19.4783544374037));
#90585=CARTESIAN_POINT('Ctrl Pts',(19.0605095737166,17.1152334077911,-19.4712321465482));
#90586=CARTESIAN_POINT('Ctrl Pts',(19.2001132485262,17.1459164044562,-19.4627978898593));
#90587=CARTESIAN_POINT('Ctrl Pts',(19.2117630323281,17.1485804774142,-19.4620877402309));
#90588=CARTESIAN_POINT('Ctrl Pts',(19.2282829172218,17.1525057209427,-19.4610709165965));
#90589=CARTESIAN_POINT('Ctrl Pts',(19.233172285768,17.1536858948858,-19.4607687440908));
#90590=CARTESIAN_POINT('Ctrl Pts',(19.2415875719835,17.1557489038434,-19.4602464789165));
#90591=CARTESIAN_POINT('Ctrl Pts',(19.2451155445436,17.1566234251094,-19.4600268643563));
#90592=CARTESIAN_POINT('Ctrl Pts',(19.251948857971,17.1583359729451,-19.4596001805042));
#90593=CARTESIAN_POINT('Ctrl Pts',(19.2552544339929,17.1591729015095,-19.4593931806813));
#90594=CARTESIAN_POINT('Ctrl Pts',(19.264161731883,17.1614510265473,-19.4588338179635));
#90595=CARTESIAN_POINT('Ctrl Pts',(19.2697595447368,17.162907188394,-19.4584806030637));
#90596=CARTESIAN_POINT('Ctrl Pts',(19.2904807578836,17.1683881710774,-19.457167063065));
#90597=CARTESIAN_POINT('Ctrl Pts',(19.3055649272845,17.1725575999223,-19.456198882689));
#90598=CARTESIAN_POINT('Ctrl Pts',(19.4501596590184,17.214256212632,-19.4468117091658));
#90599=CARTESIAN_POINT('Ctrl Pts',(19.5758408856351,17.263907782423,-19.4378492738161));
#90600=CARTESIAN_POINT('Ctrl Pts',(19.8385652757954,17.3979194730604,-19.4183720679032));
#90601=CARTESIAN_POINT('Ctrl Pts',(19.9725071704624,17.486632226586,-19.4079688140199));
#90602=CARTESIAN_POINT('Ctrl Pts',(20.1094644694638,17.6016105819765,-19.3970159620179));
#90603=CARTESIAN_POINT('Ctrl Pts',(20.1235891627616,17.6137903082944,-19.3958813755409));
#90604=CARTESIAN_POINT('Ctrl Pts',(20.1439336175515,17.6318075250723,-19.3942393830913));
#90605=CARTESIAN_POINT('Ctrl Pts',(20.1502816773317,17.6374982070091,-19.3937259012378));
#90606=CARTESIAN_POINT('Ctrl Pts',(20.1613680002001,17.6475579234683,-19.3928270847801));
#90607=CARTESIAN_POINT('Ctrl Pts',(20.1661209779698,17.6519105091277,-19.392441064033));
#90608=CARTESIAN_POINT('Ctrl Pts',(20.1753237741438,17.6604156518448,-19.3916922877939));
#90609=CARTESIAN_POINT('Ctrl Pts',(20.179775702215,17.6645658233437,-19.3913294364163));
#90610=CARTESIAN_POINT('Ctrl Pts',(20.1903950005449,17.674551274101,-19.3904623741943));
#90611=CARTESIAN_POINT('Ctrl Pts',(20.1965453170217,17.6804045982764,-19.389958943916));
#90612=CARTESIAN_POINT('Ctrl Pts',(20.2187278290756,17.7017717294069,-19.3881384275946));
#90613=CARTESIAN_POINT('Ctrl Pts',(20.2345501125293,17.7175020539885,-19.3868307625447));
#90614=CARTESIAN_POINT('Ctrl Pts',(20.378213301191,17.8649185441742,-19.3748614530499));
#90615=CARTESIAN_POINT('Ctrl Pts',(20.4886678815135,18.0124510933741,-19.3650341203674));
#90616=CARTESIAN_POINT('Ctrl Pts',(20.6187025237321,18.243411240363,-19.3505913375458));
#90617=CARTESIAN_POINT('Ctrl Pts',(20.6545501775305,18.3166753695062,-19.3461133563995));
#90618=CARTESIAN_POINT('Ctrl Pts',(20.7001659539281,18.4253760411333,-19.3393728575855));
#90619=CARTESIAN_POINT('Ctrl Pts',(20.7133803079529,18.459290746977,-19.3372565100043));
#90620=CARTESIAN_POINT('Ctrl Pts',(20.7282509523279,18.5005718107286,-19.3346454222987));
#90621=CARTESIAN_POINT('Ctrl Pts',(20.7307513370133,18.5076301347739,-19.3341977522896));
#90622=CARTESIAN_POINT('Ctrl Pts',(20.7345837881141,18.5186338782765,-19.3334977333009));
#90623=CARTESIAN_POINT('Ctrl Pts',(20.7359417773079,18.5225702945408,-19.333246893332));
#90624=CARTESIAN_POINT('Ctrl Pts',(20.7384409410638,18.5298845721234,-19.3327799843039));
#90625=CARTESIAN_POINT('Ctrl Pts',(20.7395851993978,18.5332613190467,-19.3325641005641));
#90626=CARTESIAN_POINT('Ctrl Pts',(20.7421556754325,18.5409104014784,-19.3320743392664));
#90627=CARTESIAN_POINT('Ctrl Pts',(20.7435767846128,18.5451843853615,-19.3318001663998));
#90628=CARTESIAN_POINT('Ctrl Pts',(20.747831065529,18.5581168284053,-19.3309690752267));
#90629=CARTESIAN_POINT('Ctrl Pts',(20.7506219526325,18.5667889402043,-19.3304097629595));
#90630=CARTESIAN_POINT('Ctrl Pts',(20.7716710779449,18.633672122517,-19.3260821477863));
#90631=CARTESIAN_POINT('Ctrl Pts',(20.7874596168193,18.6926246247417,-19.3221871938091));
#90632=CARTESIAN_POINT('Ctrl Pts',(20.8135818915649,18.8102855888011,-19.3143614751178));
#90633=CARTESIAN_POINT('Ctrl Pts',(20.8240267881588,18.8689175186693,-19.3104372340411));
#90634=CARTESIAN_POINT('Ctrl Pts',(20.84654308009,19.0357859231841,-19.2993132865357));
#90635=CARTESIAN_POINT('Ctrl Pts',(20.8527583948964,19.1446329813134,-19.2921187092348));
#90636=CARTESIAN_POINT('Ctrl Pts',(20.8490715742645,19.3283241096571,-19.2803152120503));
#90637=CARTESIAN_POINT('Ctrl Pts',(20.8436007149766,19.4030407929438,-19.2756058924345));
#90638=CARTESIAN_POINT('Ctrl Pts',(20.8318188154508,19.495952711619,-19.2698686362723));
#90639=CARTESIAN_POINT('Ctrl Pts',(20.8292078560918,19.5145554410462,-19.2687257719568));
#90640=CARTESIAN_POINT('Ctrl Pts',(20.8250486288661,19.54157182769,-19.2670740912115));
#90641=CARTESIAN_POINT('Ctrl Pts',(20.8236964789049,19.5500143521263,-19.2665590974263));
#90642=CARTESIAN_POINT('Ctrl Pts',(20.8212348510868,19.5648096380038,-19.2656585388559));
#90643=CARTESIAN_POINT('Ctrl Pts',(20.8201474306668,19.5711659096655,-19.2652722796448));
#90644=CARTESIAN_POINT('Ctrl Pts',(20.8179785384612,19.5835042332641,-19.2645236983071));
#90645=CARTESIAN_POINT('Ctrl Pts',(20.816900311501,19.5894867845792,-19.2641612772068));
#90646=CARTESIAN_POINT('Ctrl Pts',(20.8142595004653,19.6037862282353,-19.2632962914735));
#90647=CARTESIAN_POINT('Ctrl Pts',(20.8126727801019,19.6120985998363,-19.2627944988896));
#90648=CARTESIAN_POINT('Ctrl Pts',(20.8067569002731,19.6421119290861,-19.2609862281892));
#90649=CARTESIAN_POINT('Ctrl Pts',(20.8021373076979,19.6637546730658,-19.2596890037661));
#90650=CARTESIAN_POINT('Ctrl Pts',(20.7556427629015,19.8659941808761,-19.2476201577379));
#90651=CARTESIAN_POINT('Ctrl Pts',(20.6905580517034,20.0404235711714,-19.2377029326564));
#90652=CARTESIAN_POINT('Ctrl Pts',(20.5659209151493,20.275048167134,-19.2232204951948));
#90653=CARTESIAN_POINT('Ctrl Pts',(20.5242633268284,20.3437347209994,-19.2188064093679));
#90654=CARTESIAN_POINT('Ctrl Pts',(20.4583865313407,20.4396092966767,-19.2121527114519));
#90655=CARTESIAN_POINT('Ctrl Pts',(20.437207325325,20.4688052992242,-19.2100549776856));
#90656=CARTESIAN_POINT('Ctrl Pts',(20.4107559561063,20.5033754254829,-19.2074645382492));
#90657=CARTESIAN_POINT('Ctrl Pts',(20.4061863423335,20.5092825614914,-19.2070180379725));
#90658=CARTESIAN_POINT('Ctrl Pts',(20.3990230319104,20.5184420090598,-19.2063194544273));
#90659=CARTESIAN_POINT('Ctrl Pts',(20.3964507914676,20.5217111310702,-19.2060688701841));
#90660=CARTESIAN_POINT('Ctrl Pts',(20.3916557119651,20.5277684898818,-19.2056021893234));
#90661=CARTESIAN_POINT('Ctrl Pts',(20.3894354573937,20.5305586993971,-19.2053862764597));
#90662=CARTESIAN_POINT('Ctrl Pts',(20.3843911321713,20.5368651704445,-19.2048961283016));
#90663=CARTESIAN_POINT('Ctrl Pts',(20.3815628826702,20.5403780072367,-19.2046215956941));
#90664=CARTESIAN_POINT('Ctrl Pts',(20.3742318918431,20.54942416056,-19.2039107797717));
#90665=CARTESIAN_POINT('Ctrl Pts',(20.3697124091154,20.5549437502918,-19.2034733304858));
#90666=CARTESIAN_POINT('Ctrl Pts',(20.3417964580907,20.5886877606709,-19.2007765011327));
#90667=CARTESIAN_POINT('Ctrl Pts',(20.3176994848855,20.6163215236206,-19.1984709468753));
#90668=CARTESIAN_POINT('Ctrl Pts',(20.1774751337907,20.7689386467687,-19.185244461121));
#90669=CARTESIAN_POINT('Ctrl Pts',(20.0472910970754,20.8801503528965,-19.1737328748605));
#90670=CARTESIAN_POINT('Ctrl Pts',(19.82576354334,21.027267368159,-19.1564516786444));
#90671=CARTESIAN_POINT('Ctrl Pts',(19.7428804294575,21.0745823860423,-19.1503957560952));
#90672=CARTESIAN_POINT('Ctrl Pts',(19.6378355663715,21.1254783976778,-19.1432258873204));
#90673=CARTESIAN_POINT('Ctrl Pts',(19.618450936858,21.1345105560304,-19.1419224706049));
#90674=CARTESIAN_POINT('Ctrl Pts',(19.5907099067168,21.1469282756437,-19.1400843594447));
#90675=CARTESIAN_POINT('Ctrl Pts',(19.5824640980739,21.1505563489892,-19.1395413633423));
#90676=CARTESIAN_POINT('Ctrl Pts',(19.5682051620042,21.1567218037883,-19.1386081126469));
#90677=CARTESIAN_POINT('Ctrl Pts',(19.5622030468134,21.1592841950755,-19.1382170076031));
#90678=CARTESIAN_POINT('Ctrl Pts',(19.5506923942465,21.1641354571764,-19.1374702370996));
#90679=CARTESIAN_POINT('Ctrl Pts',(19.5451858531175,21.1664288771835,-19.137114419822));
#90680=CARTESIAN_POINT('Ctrl Pts',(19.5308511744754,21.1723281576335,-19.13619181492));
#90681=CARTESIAN_POINT('Ctrl Pts',(19.5220081726605,21.1758977226645,-19.135626259429));
#90682=CARTESIAN_POINT('Ctrl Pts',(19.4918209366287,21.1878465295343,-19.1337075895897));
#90683=CARTESIAN_POINT('Ctrl Pts',(19.4703643509266,21.1959388848163,-19.1323641064201));
#90684=CARTESIAN_POINT('Ctrl Pts',(19.2828328255767,21.2632069240264,-19.1207863792827));
#90685=CARTESIAN_POINT('Ctrl Pts',(19.1101028362507,21.3017711607132,-19.111311225342));
#90686=CARTESIAN_POINT('Ctrl Pts',(18.8485351998096,21.3266656020323,-19.0970128830124));
#90687=CARTESIAN_POINT('Ctrl Pts',(18.7620791686531,21.3295769870634,-19.0922794517899));
#90688=CARTESIAN_POINT('Ctrl Pts',(18.6380316834745,21.3261592573976,-19.0851932757912));
#90689=CARTESIAN_POINT('Ctrl Pts',(18.600405371339,21.3241163437425,-19.0830044483095));
#90690=CARTESIAN_POINT('Ctrl Pts',(18.5553176942743,21.3204593710859,-19.0803129943747));
#90691=CARTESIAN_POINT('Ctrl Pts',(18.5477825347966,21.3198075437039,-19.0798608844819));
#90692=CARTESIAN_POINT('Ctrl Pts',(18.536088244582,21.3187327661038,-19.0791554184968));
#90693=CARTESIAN_POINT('Ctrl Pts',(18.5319265135599,21.3183378423083,-19.0789036095811));
#90694=CARTESIAN_POINT('Ctrl Pts',(18.5242190331953,21.3175834062839,-19.0784358280959));
#90695=CARTESIAN_POINT('Ctrl Pts',(18.5206730117286,21.3172272662644,-19.0782200467525));
#90696=CARTESIAN_POINT('Ctrl Pts',(18.5126690199395,21.3164029756263,-19.0777317151874));
#90697=CARTESIAN_POINT('Ctrl Pts',(18.5082116527515,21.3159296220783,-19.0774588771022));
#90698=CARTESIAN_POINT('Ctrl Pts',(18.4950908913945,21.3144940975508,-19.0766531945077));
#90699=CARTESIAN_POINT('Ctrl Pts',(18.4864320204656,21.3134925850316,-19.0761182152909));
#90700=CARTESIAN_POINT('Ctrl Pts',(18.4248765576603,21.3059873631538,-19.0722929152636));
#90701=CARTESIAN_POINT('Ctrl Pts',(18.3722404125648,21.2975421926583,-19.0689057101185));
#90702=CARTESIAN_POINT('Ctrl Pts',(18.3023591118912,21.2836066042052,-19.0643005755572));
#90703=CARTESIAN_POINT('Ctrl Pts',(18.2847799797367,21.2798676467466,-19.06313281346));
#90704=CARTESIAN_POINT('Ctrl Pts',(18.2202261468215,21.265275966019,-19.0588147822249));
#90705=CARTESIAN_POINT('Ctrl Pts',(18.1735793185627,21.2530435215245,-19.055636509265));
#90706=CARTESIAN_POINT('Ctrl Pts',(18.0225990922783,21.2078879835835,-19.0452266626765));
#90707=CARTESIAN_POINT('Ctrl Pts',(17.9203845661018,21.1684693515016,-19.0379941040625));
#90708=CARTESIAN_POINT('Ctrl Pts',(17.7533800121832,21.0887114999822,-19.0260981524289));
#90709=CARTESIAN_POINT('Ctrl Pts',(17.6868830898271,21.0524571441374,-19.0213353713156));
#90710=CARTESIAN_POINT('Ctrl Pts',(17.6063835888865,21.0027944167638,-19.0155404392381));
#90711=CARTESIAN_POINT('Ctrl Pts',(17.5904361816114,20.9926587305555,-19.0143907453355));
#90712=CARTESIAN_POINT('Ctrl Pts',(17.5674553637061,20.977617123585,-19.0127310771272));
#90713=CARTESIAN_POINT('Ctrl Pts',(17.5603130238832,20.9728800570067,-19.012214841149));
#90714=CARTESIAN_POINT('Ctrl Pts',(17.5478447021397,20.9645011358771,-19.0113128492244));
#90715=CARTESIAN_POINT('Ctrl Pts',(17.5425062727328,20.9608780881755,-19.0109263920377));
#90716=CARTESIAN_POINT('Ctrl Pts',(17.5321751552666,20.9537974416274,-19.0101779623279));
#90717=CARTESIAN_POINT('Ctrl Pts',(17.5271806240426,20.9503426559933,-19.0098158883146));
#90718=CARTESIAN_POINT('Ctrl Pts',(17.515280773985,20.9420354345628,-19.0089525815475));
#90719=CARTESIAN_POINT('Ctrl Pts',(17.5083894362443,20.9371630794093,-19.0084521139712));
#90720=CARTESIAN_POINT('Ctrl Pts',(17.4836527635305,20.919450788915,-19.0066536159706));
#90721=CARTESIAN_POINT('Ctrl Pts',(17.4659781666797,20.9063739981265,-19.0053647071586));
#90722=CARTESIAN_POINT('Ctrl Pts',(17.3000937186315,20.7795964859562,-18.9932203634322));
#90723=CARTESIAN_POINT('Ctrl Pts',(17.1673457687471,20.6470301461303,-18.9832348352213));
#90724=CARTESIAN_POINT('Ctrl Pts',(17.005442473164,20.435775045624,-18.9687214714853));
#90725=CARTESIAN_POINT('Ctrl Pts',(16.9607585652638,20.3701366989198,-18.9643555312532));
#90726=CARTESIAN_POINT('Ctrl Pts',(16.9014073589746,20.2714602486633,-18.9577673299044));
#90727=CARTESIAN_POINT('Ctrl Pts',(16.8837304152689,20.2403074603536,-18.9556837525783));
#90728=CARTESIAN_POINT('Ctrl Pts',(16.8633406754344,20.2021499590242,-18.9531090196168));
#90729=CARTESIAN_POINT('Ctrl Pts',(16.8598628565168,20.1955580295374,-18.9526634172904));
#90730=CARTESIAN_POINT('Ctrl Pts',(16.8544998952484,20.1852615832054,-18.9519659357869));
#90731=CARTESIAN_POINT('Ctrl Pts',(16.8525906925139,20.1815695715885,-18.9517155479896));
#90732=CARTESIAN_POINT('Ctrl Pts',(16.8490636468279,20.1746994667743,-18.951249041803));
#90733=CARTESIAN_POINT('Ctrl Pts',(16.8474429569923,20.1715228995918,-18.9510331059631));
#90734=CARTESIAN_POINT('Ctrl Pts',(16.8437888032994,20.1643157986354,-18.9505426578842));
#90735=CARTESIAN_POINT('Ctrl Pts',(16.8417602110571,20.160282866341,-18.9502678467809));
#90736=CARTESIAN_POINT('Ctrl Pts',(16.8357860253825,20.1483106776904,-18.9494510231292));
#90737=CARTESIAN_POINT('Ctrl Pts',(16.831877445271,20.1403532054228,-18.9489067885678));
#90738=CARTESIAN_POINT('Ctrl Pts',(16.8031431866498,20.0809125291191,-18.9448329616298));
#90739=CARTESIAN_POINT('Ctrl Pts',(16.7803637992109,20.0284718308009,-18.9411920268991));
#90740=CARTESIAN_POINT('Ctrl Pts',(16.6996314188873,19.8198990120479,-18.9267029874953));
#90741=CARTESIAN_POINT('Ctrl Pts',(16.6580537897843,19.6580665212596,-18.9155001378934));
#90742=CARTESIAN_POINT('Ctrl Pts',(16.6280919355396,19.435161618524,-18.9010061673904));
#90743=CARTESIAN_POINT('Ctrl Pts',(16.6227108983252,19.3770015101593,-18.8973011305402));
#90744=CARTESIAN_POINT('Ctrl Pts',(16.617921324783,19.2829677512959,-18.8914414386409));
#90745=CARTESIAN_POINT('Ctrl Pts',(16.6170073710065,19.2472045679689,-18.8892429310058));
#90746=CARTESIAN_POINT('Ctrl Pts',(16.6169977968346,19.2004601970563,-18.8864068441664));
#90747=CARTESIAN_POINT('Ctrl Pts',(16.6170808697125,19.189486781312,-18.8857437475015));
#90748=CARTESIAN_POINT('Ctrl Pts',(16.617355670881,19.1715808612138,-18.8846659982215));
#90749=CARTESIAN_POINT('Ctrl Pts',(16.6174961452151,19.1646478807895,-18.8842497477679));
#90750=CARTESIAN_POINT('Ctrl Pts',(16.6178328488804,19.1512748012638,-18.8834488079317));
#90751=CARTESIAN_POINT('Ctrl Pts',(16.6180244184906,19.1448346713578,-18.883063977102));
#90752=CARTESIAN_POINT('Ctrl Pts',(16.6185373485299,19.1298874778342,-18.8821728055198));
#90753=CARTESIAN_POINT('Ctrl Pts',(16.6188806293354,19.1213812403198,-18.8816671568674));
#90754=CARTESIAN_POINT('Ctrl Pts',(16.620136566495,19.0943135080247,-18.8800627596263));
#90755=CARTESIAN_POINT('Ctrl Pts',(16.6212423368925,19.0757615346521,-18.8789700616719));
#90756=CARTESIAN_POINT('Ctrl Pts',(16.6243860730752,19.0325961609319,-18.8764423806009));
#90757=CARTESIAN_POINT('Ctrl Pts',(16.6266107500515,19.007998839698,-18.8750132004309));
#90758=CARTESIAN_POINT('Ctrl Pts',(16.6359173607672,18.9219186647825,-18.8700446062002));
#90759=CARTESIAN_POINT('Ctrl Pts',(16.6452642980639,18.8607103928403,-18.8665717730464));
#90760=CARTESIAN_POINT('Ctrl Pts',(16.678497031111,18.6927922113537,-18.857102765276));
#90761=CARTESIAN_POINT('Ctrl Pts',(16.7079721274187,18.5874456088998,-18.8512347675934));
#90762=CARTESIAN_POINT('Ctrl Pts',(16.7454194035981,18.4848896698064,-18.845275399947));
#90763=CARTESIAN_POINT('Origin',(18.734,19.211,0.));
#90764=CARTESIAN_POINT('',(16.7454193875989,18.4848897136231,-18.0457833433865));
#90765=CARTESIAN_POINT('',(16.7454194512262,18.4848895393686,-18.2676549287063));
#90766=CARTESIAN_POINT('',(16.7454194503191,18.4848895418526,0.));
#90767=CARTESIAN_POINT('',(16.6170000023184,19.2110990761722,-18.3109437209775));
#90768=CARTESIAN_POINT('Ctrl Pts',(16.7454194512262,18.4848895393686,-18.2676549287063));
#90769=CARTESIAN_POINT('Ctrl Pts',(16.7422625743728,18.493535199011,-18.2681689766162));
#90770=CARTESIAN_POINT('Ctrl Pts',(16.7391619133878,18.5022019024759,-18.2686817414929));
#90771=CARTESIAN_POINT('Ctrl Pts',(16.7026446946734,18.6064098304461,-18.2748185764456));
#90772=CARTESIAN_POINT('Ctrl Pts',(16.6760643065157,18.7042108460221,-18.2802824916259));
#90773=CARTESIAN_POINT('Ctrl Pts',(16.6332961709258,18.9222616774293,-18.292365115819));
#90774=CARTESIAN_POINT('Ctrl Pts',(16.62023343224,19.0427466454246,-18.2989795629078));
#90775=CARTESIAN_POINT('Ctrl Pts',(16.6172718865579,19.1751735243589,-18.3067857740772));
#90776=CARTESIAN_POINT('Ctrl Pts',(16.6171084113102,19.1866806408802,-18.3074685689643));
#90777=CARTESIAN_POINT('Ctrl Pts',(16.6170172097224,19.2017503970018,-18.3083692892897));
#90778=CARTESIAN_POINT('Ctrl Pts',(16.6170046428134,19.2053125820636,-18.3085826791177));
#90779=CARTESIAN_POINT('Ctrl Pts',(16.6170002820809,19.2096563900998,-18.3088434923776));
#90780=CARTESIAN_POINT('Ctrl Pts',(16.6169999302933,19.2104380262339,-18.3088904475228));
#90781=CARTESIAN_POINT('Ctrl Pts',(16.617000011396,19.2112196607865,-18.3089374264593));
#90782=CARTESIAN_POINT('Ctrl Pts',(16.6170000023184,19.2110990761722,-18.3109437209775));
#90783=CARTESIAN_POINT('Ctrl Pts',(16.6170002492315,19.2163749670546,-18.3112630160645));
#90784=CARTESIAN_POINT('Ctrl Pts',(16.6170202186042,19.2216508039048,-18.3115823111514));
#90785=CARTESIAN_POINT('Ctrl Pts',(16.6170599094811,19.2269264921969,-18.3119016062384));
#90786=CARTESIAN_POINT('Ctrl Pts',(16.6176053981758,19.2994325325996,-18.3162898151688));
#90787=CARTESIAN_POINT('Ctrl Pts',(16.6218813020779,19.3720520465351,-18.3206780240992));
#90788=CARTESIAN_POINT('Ctrl Pts',(16.6299021760198,19.4443695505458,-18.3250662330295));
#90789=CARTESIAN_POINT('Ctrl Pts',(16.6379111456549,19.5165797233901,-18.3294479291303));
#90790=CARTESIAN_POINT('Ctrl Pts',(16.6496539988947,19.588488300638,-18.333829625231));
#90791=CARTESIAN_POINT('Ctrl Pts',(16.6650932824124,19.6596802802897,-18.3382113213318));
#90792=CARTESIAN_POINT('Ctrl Pts',(16.6805144235432,19.7307886036996,-18.3425878685909));
#90793=CARTESIAN_POINT('Ctrl Pts',(16.6996232646346,19.8011815331899,-18.3469644158501));
#90794=CARTESIAN_POINT('Ctrl Pts',(16.7223308201356,19.8704513710532,-18.3513409631092));
#90795=CARTESIAN_POINT('Ctrl Pts',(16.745023974835,19.939677278992,-18.3557147348257));
#90796=CARTESIAN_POINT('Ctrl Pts',(16.7713111657671,20.0077810512476,-18.3600885065421));
#90797=CARTESIAN_POINT('Ctrl Pts',(16.8010531665407,20.0743687155669,-18.3644622782586));
#90798=CARTESIAN_POINT('Ctrl Pts',(16.8307861167235,20.1409361170363,-18.3688347190217));
#90799=CARTESIAN_POINT('Ctrl Pts',(16.8639715929647,20.20598788633,-18.3732071597847));
#90800=CARTESIAN_POINT('Ctrl Pts',(16.9004223233179,20.269150227318,-18.3775796005477));
#90801=CARTESIAN_POINT('Ctrl Pts',(16.9368739857203,20.332314183374,-18.3819521531146));
#90802=CARTESIAN_POINT('Ctrl Pts',(16.9765908251609,20.3935881984058,-18.3863247056814));
#90803=CARTESIAN_POINT('Ctrl Pts',(17.019340565139,20.452624751059,-18.3906972582483));
#90804=CARTESIAN_POINT('Ctrl Pts',(17.0621346724099,20.5117225740734,-18.3950743488151));
#90805=CARTESIAN_POINT('Ctrl Pts',(17.10796768121,20.5685779068979,-18.399451439382));
#90806=CARTESIAN_POINT('Ctrl Pts',(17.156565568357,20.6228745035828,-18.4038285299488));
#90807=CARTESIAN_POINT('Ctrl Pts',(17.205189996614,20.6772007536545,-18.4082080110073));
#90808=CARTESIAN_POINT('Ctrl Pts',(17.2565819695238,20.7289651427766,-18.4125874920657));
#90809=CARTESIAN_POINT('Ctrl Pts',(17.3104308762819,20.7778886208013,-18.4169669731242));
#90810=CARTESIAN_POINT('Ctrl Pts',(17.364375229866,20.8268988153625,-18.4213542167834));
#90811=CARTESIAN_POINT('Ctrl Pts',(17.4207848402039,20.8730577373945,-18.4257414604427));
#90812=CARTESIAN_POINT('Ctrl Pts',(17.4793168103114,20.9161272953985,-18.430128704102));
#90813=CARTESIAN_POINT('Ctrl Pts',(17.5191129099216,20.9454104447157,-18.4331116070413));
#90814=CARTESIAN_POINT('Ctrl Pts',(17.5598894741973,20.9732663668681,-18.4360945099806));
#90815=CARTESIAN_POINT('Ctrl Pts',(17.6015321394767,20.9996323112596,-18.4390774129199));
#90816=CARTESIAN_POINT('Ctrl Pts',(17.6627935078072,21.0384197860744,-18.4434656218502));
#90817=CARTESIAN_POINT('Ctrl Pts',(17.7261694924202,21.0741319931223,-18.4478538307805));
#90818=CARTESIAN_POINT('Ctrl Pts',(17.791318615734,21.1065318007774,-18.4522420397107));
#90819=CARTESIAN_POINT('Ctrl Pts',(17.8563710469468,21.1388835217458,-18.4566237358114));
#90820=CARTESIAN_POINT('Ctrl Pts',(17.9231909643681,21.1679323895269,-18.461005431912));
#90821=CARTESIAN_POINT('Ctrl Pts',(17.9914091442161,21.1934852637299,-18.4653871280127));
#90822=CARTESIAN_POINT('Ctrl Pts',(18.0595471622737,21.2190081112721,-18.4697636752717));
#90823=CARTESIAN_POINT('Ctrl Pts',(18.1290797293043,21.2410429575788,-18.4741402225307));
#90824=CARTESIAN_POINT('Ctrl Pts',(18.1996158698647,21.2594439463797,-18.4785167697897));
#90825=CARTESIAN_POINT('Ctrl Pts',(18.2701072774298,21.2778332655408,-18.482890541506));
#90826=CARTESIAN_POINT('Ctrl Pts',(18.3416005301136,21.2925931782368,-18.4872643132223));
#90827=CARTESIAN_POINT('Ctrl Pts',(18.4136889989941,21.3036275021213,-18.4916380849387));
#90828=CARTESIAN_POINT('Ctrl Pts',(18.4857555311113,21.314658468224,-18.4960105257016));
#90829=CARTESIAN_POINT('Ctrl Pts',(18.558416443296,21.3219660233356,-18.5003829664645));
#90830=CARTESIAN_POINT('Ctrl Pts',(18.6312560654046,21.3255053047708,-18.5047554072274));
#90831=CARTESIAN_POINT('Ctrl Pts',(18.7040975500302,21.3290446767058,-18.5091279597941));
#90832=CARTESIAN_POINT('Ctrl Pts',(18.7771172717461,21.3288155622467,-18.5135005123608));
#90833=CARTESIAN_POINT('Ctrl Pts',(18.8498972932253,21.3248251624538,-18.5178730649275));
#90834=CARTESIAN_POINT('Ctrl Pts',(18.922752848556,21.3208306212736,-18.5222501554941));
#90835=CARTESIAN_POINT('Ctrl Pts',(18.9953677242794,21.3130670274164,-18.5266272460608));
#90836=CARTESIAN_POINT('Ctrl Pts',(19.0673276840476,21.3015936130792,-18.5310043366275));
#90837=CARTESIAN_POINT('Ctrl Pts',(19.1393269438205,21.2901139326845,-18.5353838176858));
#90838=CARTESIAN_POINT('Ctrl Pts',(19.2106701033884,21.274920498468,-18.5397632987441));
#90839=CARTESIAN_POINT('Ctrl Pts',(19.2809543980001,21.2561234404085,-18.5441427798024));
#90840=CARTESIAN_POINT('Ctrl Pts',(19.3513632710524,21.2372930646897,-18.5485300234614));
#90841=CARTESIAN_POINT('Ctrl Pts',(19.4207090718549,21.2148464584352,-18.5529172671205));
#90842=CARTESIAN_POINT('Ctrl Pts',(19.4886059995023,21.1889430693312,-18.5573045107796));
#90843=CARTESIAN_POINT('Ctrl Pts',(19.5347693678655,21.1713312607487,-18.5602874137202));
#90844=CARTESIAN_POINT('Ctrl Pts',(19.5802633709739,21.1521225055481,-18.5632703166607));
#90845=CARTESIAN_POINT('Ctrl Pts',(19.624973342625,21.1313789997632,-18.5662532196012));
#90846=CARTESIAN_POINT('Ctrl Pts',(19.690747087515,21.1008628082464,-18.5706414285353));
#90847=CARTESIAN_POINT('Ctrl Pts',(19.7550796205674,21.0669039749609,-18.5750296374695));
#90848=CARTESIAN_POINT('Ctrl Pts',(19.8175867162729,21.0296612736617,-18.5794178464036));
#90849=CARTESIAN_POINT('Ctrl Pts',(19.8800010410847,20.9924738467062,-18.583799542508));
#90850=CARTESIAN_POINT('Ctrl Pts',(19.9405948958109,20.9520124717685,-18.5881812386125));
#90851=CARTESIAN_POINT('Ctrl Pts',(19.9990060261175,20.9084830643887,-18.592562934717));
#90852=CARTESIAN_POINT('Ctrl Pts',(20.0573485186974,20.8650048075267,-18.5969394819799));
#90853=CARTESIAN_POINT('Ctrl Pts',(20.113512997131,20.818465966753,-18.6013160292427));
#90854=CARTESIAN_POINT('Ctrl Pts',(20.1671651917848,20.7691163413097,-18.6056925765056));
#90855=CARTESIAN_POINT('Ctrl Pts',(20.2207833609965,20.7197980126817,-18.6100663482258));
#90856=CARTESIAN_POINT('Ctrl Pts',(20.2718920534931,20.6676727619683,-18.6144401199459));
#90857=CARTESIAN_POINT('Ctrl Pts',(20.3201902946191,20.6130304380634,-18.6188138916661));
#90858=CARTESIAN_POINT('Ctrl Pts',(20.368473838428,20.5584047420012,-18.6231863324329));
#90859=CARTESIAN_POINT('Ctrl Pts',(20.4139483094877,20.5012638546127,-18.6275587731996));
#90860=CARTESIAN_POINT('Ctrl Pts',(20.4563509910144,20.4419330053873,-18.6319312139664));
#90861=CARTESIAN_POINT('Ctrl Pts',(20.4987547567822,20.3826006390657,-18.6363037665369));
#90862=CARTESIAN_POINT('Ctrl Pts',(20.5380862982191,20.3210785933454,-18.6406763191075));
#90863=CARTESIAN_POINT('Ctrl Pts',(20.574125448729,20.2577221851762,-18.645048871678));
#90864=CARTESIAN_POINT('Ctrl Pts',(20.6102020020282,20.1943000233375,-18.6494259622485));
#90865=CARTESIAN_POINT('Ctrl Pts',(20.6429791031792,20.1290401182302,-18.6538030528189));
#90866=CARTESIAN_POINT('Ctrl Pts',(20.6722823388071,20.0623228383337,-18.6581801433894));
#90867=CARTESIAN_POINT('Ctrl Pts',(20.7016015780193,19.9955691216548,-18.6625596244515));
#90868=CARTESIAN_POINT('Ctrl Pts',(20.7274430033785,19.9273568969102,-18.6669391055136));
#90869=CARTESIAN_POINT('Ctrl Pts',(20.7496812078475,19.858084436786,-18.6713185865756));
#90870=CARTESIAN_POINT('Ctrl Pts',(20.7719588293842,19.7886891916923,-18.6757058302384));
#90871=CARTESIAN_POINT('Ctrl Pts',(20.7906203524689,19.7182304251234,-18.6800930739012));
#90872=CARTESIAN_POINT('Ctrl Pts',(20.8055910206596,19.6471188405955,-18.684480317564));
#90873=CARTESIAN_POINT('Ctrl Pts',(20.8157696323546,19.5987698159095,-18.6874632204702));
#90874=CARTESIAN_POINT('Ctrl Pts',(20.8242431499881,19.5501192245651,-18.6904461233765));
#90875=CARTESIAN_POINT('Ctrl Pts',(20.8310018039417,19.501297148221,-18.6934290262827));
#90876=CARTESIAN_POINT('Ctrl Pts',(20.8409445967655,19.4294740021259,-18.6978172352092));
#90877=CARTESIAN_POINT('Ctrl Pts',(20.8472125720512,19.3569992504144,-18.7022054441356));
#90878=CARTESIAN_POINT('Ctrl Pts',(20.8497312594192,19.2842819071557,-18.7065936530621));
#90879=CARTESIAN_POINT('Ctrl Pts',(20.8522462086376,19.211672488491,-18.7109753491589));
#90880=CARTESIAN_POINT('Ctrl Pts',(20.8510228997993,19.1388216711234,-18.7153570452558));
#90881=CARTESIAN_POINT('Ctrl Pts',(20.8460383938856,19.0661455117948,-18.7197387413526));
#90882=CARTESIAN_POINT('Ctrl Pts',(20.841059745163,18.9935547527367,-18.7241152886079));
#90883=CARTESIAN_POINT('Ctrl Pts',(20.8323287119819,18.9211387228713,-18.7284918358632));
#90884=CARTESIAN_POINT('Ctrl Pts',(20.8198744021603,18.8493137016523,-18.7328683831184));
#90885=CARTESIAN_POINT('Ctrl Pts',(20.8074279906809,18.7775342308174,-18.7372421548311));
#90886=CARTESIAN_POINT('Ctrl Pts',(20.7912630697938,18.7063454990751,-18.7416159265437));
#90887=CARTESIAN_POINT('Ctrl Pts',(20.7714604446762,18.6361574681881,-18.7459896982563));
#90888=CARTESIAN_POINT('Ctrl Pts',(20.7516638455637,18.5659907957541,-18.7503621390155));
#90889=CARTESIAN_POINT('Ctrl Pts',(20.7282318707929,18.4968246835911,-18.7547345797748));
#90890=CARTESIAN_POINT('Ctrl Pts',(20.7012957832832,18.4290560754913,-18.759107020534));
#90891=CARTESIAN_POINT('Ctrl Pts',(20.6743590070145,18.3612857345401,-18.7634795730971));
#90892=CARTESIAN_POINT('Ctrl Pts',(20.6439181201446,18.2949134161269,-18.7678521256601));
#90893=CARTESIAN_POINT('Ctrl Pts',(20.6101527159951,18.2303165718418,-18.7722246782232));
#90894=CARTESIAN_POINT('Ctrl Pts',(20.5763522688349,18.1656526865138,-18.7766017687863));
#90895=CARTESIAN_POINT('Ctrl Pts',(20.5392206395554,18.1027683827099,-18.7809788593495));
#90896=CARTESIAN_POINT('Ctrl Pts',(20.4989832512009,18.0420162007194,-18.7853559499126));
#90897=CARTESIAN_POINT('Ctrl Pts',(20.4587238877147,17.9812308397069,-18.7897354309674));
#90898=CARTESIAN_POINT('Ctrl Pts',(20.4153556750912,17.9225803070075,-18.7941149120222));
#90899=CARTESIAN_POINT('Ctrl Pts',(20.3691456171801,17.8663856275434,-18.798494393077));
#90900=CARTESIAN_POINT('Ctrl Pts',(20.3228536522502,17.8100913433856,-18.8028816367327));
#90901=CARTESIAN_POINT('Ctrl Pts',(20.2737101085662,17.7562619617535,-18.8072688803884));
#90902=CARTESIAN_POINT('Ctrl Pts',(20.2220198585452,17.7051826470069,-18.8116561240441));
#90903=CARTESIAN_POINT('Ctrl Pts',(20.1868754689052,17.6704536344897,-18.8146390270175));
#90904=CARTESIAN_POINT('Ctrl Pts',(20.1505545743004,17.6369951039851,-18.8176219299908));
#90905=CARTESIAN_POINT('Ctrl Pts',(20.1131612647178,17.6048856809361,-18.8206048329642));
#90906=CARTESIAN_POINT('Ctrl Pts',(20.0581512102737,17.5576488589,-18.8249930418924));
#90907=CARTESIAN_POINT('Ctrl Pts',(20.0006041495888,17.5131492751,-18.8293812508206));
#90908=CARTESIAN_POINT('Ctrl Pts',(19.9408236893632,17.4716709388986,-18.8337694597489));
#90909=CARTESIAN_POINT('Ctrl Pts',(19.8811319532531,17.4302541634259,-18.8381511558474));
#90910=CARTESIAN_POINT('Ctrl Pts',(19.8192137908503,17.3918500068481,-18.842532851946));
#90911=CARTESIAN_POINT('Ctrl Pts',(19.7554066235765,17.3567029608733,-18.8469145480445));
#90912=CARTESIAN_POINT('Ctrl Pts',(19.6916744348034,17.3215972154753,-18.8512910953013));
#90913=CARTESIAN_POINT('Ctrl Pts',(19.6260580710909,17.2897412091782,-18.8556676425582));
#90914=CARTESIAN_POINT('Ctrl Pts',(19.5589233130916,17.2613357910866,-18.860044189815));
#90915=CARTESIAN_POINT('Ctrl Pts',(19.4918311309807,17.2329483872986,-18.8644179615291));
#90916=CARTESIAN_POINT('Ctrl Pts',(19.4232229083437,17.2080074173232,-18.8687917332433));
#90917=CARTESIAN_POINT('Ctrl Pts',(19.353487096455,17.1866668413214,-18.8731655049574));
#90918=CARTESIAN_POINT('Ctrl Pts',(19.2837725054087,17.1653327593287,-18.8775379457181));
#90919=CARTESIAN_POINT('Ctrl Pts',(19.2129314673135,17.1475970372528,-18.8819103864788));
#90920=CARTESIAN_POINT('Ctrl Pts',(19.1413687992098,17.1335641618981,-18.8862828272394));
#90921=CARTESIAN_POINT('Ctrl Pts',(19.0698043012414,17.1195309277212,-18.8906553798039));
#90922=CARTESIAN_POINT('Ctrl Pts',(18.9975186103768,17.1092008191083,-18.8950279323683));
#90923=CARTESIAN_POINT('Ctrl Pts',(18.9249263141292,17.1026271338843,-18.8994004849327));
#90924=CARTESIAN_POINT('Ctrl Pts',(18.8522586788588,17.0960466262418,-18.9037775754971));
#90925=CARTESIAN_POINT('Ctrl Pts',(18.7792842843242,17.093230369319,-18.9081546660615));
#90926=CARTESIAN_POINT('Ctrl Pts',(18.7064215783365,17.0941796413823,-18.9125317566259));
#90927=CARTESIAN_POINT('Ctrl Pts',(18.6335190793211,17.0951294318782,-18.9169112376818));
#90928=CARTESIAN_POINT('Ctrl Pts',(18.5607288719984,17.0998488145903,-18.9212907187378));
#90929=CARTESIAN_POINT('Ctrl Pts',(18.4884654116445,17.1082870462374,-18.9256701997938));
#90930=CARTESIAN_POINT('Ctrl Pts',(18.4160738647923,17.1167402345934,-18.9300574434505));
#90931=CARTESIAN_POINT('Ctrl Pts',(18.3442114053892,17.1289253543984,-18.9344446871073));
#90932=CARTESIAN_POINT('Ctrl Pts',(18.2732828331912,17.1447404102563,-18.938831930764));
#90933=CARTESIAN_POINT('Ctrl Pts',(18.2250582383096,17.1554931244045,-18.9418148337245));
#90934=CARTESIAN_POINT('Ctrl Pts',(18.1772650979153,17.1679227808449,-18.9447977366851));
#90935=CARTESIAN_POINT('Ctrl Pts',(18.1300258654972,17.1819844148327,-18.9477806396456));
#90936=CARTESIAN_POINT('Ctrl Pts',(18.0605280442512,17.2026717307626,-18.9521690525416));
#90937=CARTESIAN_POINT('Ctrl Pts',(17.9919586602192,17.2269742190354,-18.9565574654377));
#90938=CARTESIAN_POINT('Ctrl Pts',(17.9247209128519,17.2547903079923,-18.9609458783337));
#90939=CARTESIAN_POINT('Ctrl Pts',(17.8574469481214,17.2826213799824,-18.9653366550321));
#90940=CARTESIAN_POINT('Ctrl Pts',(17.7915065313946,17.3139697419478,-18.9697274317305));
#90941=CARTESIAN_POINT('Ctrl Pts',(17.7272902810914,17.3486830178901,-18.9741182084289));
#90942=CARTESIAN_POINT('Ctrl Pts',(17.6632831696942,17.3832832399478,-18.9784946852852));
#90943=CARTESIAN_POINT('Ctrl Pts',(17.6009894540069,17.4212262970143,-18.9828711621416));
#90944=CARTESIAN_POINT('Ctrl Pts',(17.5407759394806,17.4623132523526,-18.987247638998));
#90945=CARTESIAN_POINT('Ctrl Pts',(17.4806016975384,17.5033734098712,-18.9916212614194));
#90946=CARTESIAN_POINT('Ctrl Pts',(17.4225053615492,17.5475731249768,-18.9959948838409));
#90947=CARTESIAN_POINT('Ctrl Pts',(17.3668265524039,17.5946690424953,-19.0003685062624));
#90948=CARTESIAN_POINT('Ctrl Pts',(17.3111656907014,17.6417497791703,-19.0047407188955));
#90949=CARTESIAN_POINT('Ctrl Pts',(17.2579211760136,17.691724552697,-19.0091129315286));
#90950=CARTESIAN_POINT('Ctrl Pts',(17.2073998648577,17.7443094984342,-19.0134851441618));
#90951=CARTESIAN_POINT('Ctrl Pts',(17.1565195530969,17.7972681088071,-19.0178884254062));
#90952=CARTESIAN_POINT('Ctrl Pts',(17.1084016692992,17.8528738026132,-19.0222917066506));
#90953=CARTESIAN_POINT('Ctrl Pts',(17.0633209239241,17.9107998520373,-19.0266949878951));
#90954=CARTESIAN_POINT('Ctrl Pts',(17.0185206472328,17.9683655160528,-19.0310708742399));
#90955=CARTESIAN_POINT('Ctrl Pts',(16.9767200693617,18.0282223204899,-19.0354467605847));
#90956=CARTESIAN_POINT('Ctrl Pts',(16.9381461792585,18.0900191551467,-19.0398226469295));
#90957=CARTESIAN_POINT('Ctrl Pts',(16.8992100558504,18.1523963012936,-19.0442396256237));
#90958=CARTESIAN_POINT('Ctrl Pts',(16.8635617990236,18.2167496759085,-19.048656604318));
#90959=CARTESIAN_POINT('Ctrl Pts',(16.8313871440048,18.2826933048815,-19.0530735830123));
#90960=CARTESIAN_POINT('Ctrl Pts',(16.799212488986,18.3486369338544,-19.0574905617065));
#90961=CARTESIAN_POINT('Ctrl Pts',(16.7705115861154,18.4161703371716,-19.0619075404008));
#90962=CARTESIAN_POINT('Ctrl Pts',(16.7454194503191,18.4848895418526,-19.066324519095));
#90963=CARTESIAN_POINT('',(16.6170009086255,19.2090541496144,-18.089014757963));
#90964=CARTESIAN_POINT('Ctrl Pts',(16.7454194035981,18.4848896698064,-18.845275399947));
#90965=CARTESIAN_POINT('Ctrl Pts',(16.7566881830226,18.4540281392966,-18.8434820839473));
#90966=CARTESIAN_POINT('Ctrl Pts',(16.7686788833216,18.4234193640937,-18.8416796887102));
#90967=CARTESIAN_POINT('Ctrl Pts',(16.8104693873181,18.3236520192083,-18.8356907737385));
#90968=CARTESIAN_POINT('Ctrl Pts',(16.8432351033399,18.2558235694364,-18.8314361934986));
#90969=CARTESIAN_POINT('Ctrl Pts',(16.8841144410632,18.1815815125323,-18.826413132321));
#90970=CARTESIAN_POINT('Ctrl Pts',(16.8887460985814,18.1733020501008,-18.8258476348406));
#90971=CARTESIAN_POINT('Ctrl Pts',(16.8956954523512,18.1610731661099,-18.8250040399154));
#90972=CARTESIAN_POINT('Ctrl Pts',(16.8979706398703,18.1570995520131,-18.8247286083055));
#90973=CARTESIAN_POINT('Ctrl Pts',(16.9020434466171,18.1500396127087,-18.8242368429802));
#90974=CARTESIAN_POINT('Ctrl Pts',(16.9038360024033,18.1469504247672,-18.8240208375938));
#90975=CARTESIAN_POINT('Ctrl Pts',(16.9077088758036,18.1403148765687,-18.8235550653782));
#90976=CARTESIAN_POINT('Ctrl Pts',(16.9097916788551,18.136770087804,-18.823305142465));
#90977=CARTESIAN_POINT('Ctrl Pts',(16.9155744855488,18.1269934619521,-18.8226128477397));
#90978=CARTESIAN_POINT('Ctrl Pts',(16.919296144699,18.1207745920248,-18.8221691015424));
#90979=CARTESIAN_POINT('Ctrl Pts',(16.9399459720041,18.0866675486583,-18.8197172761966));
#90980=CARTESIAN_POINT('Ctrl Pts',(16.9574841398768,18.0591560678372,-18.8176726580399));
#90981=CARTESIAN_POINT('Ctrl Pts',(17.0662168418627,17.8969844598258,-18.8052647618544));
#90982=CARTESIAN_POINT('Ctrl Pts',(17.1720442315182,17.7727956955694,-18.7943129863953));
#90983=CARTESIAN_POINT('Ctrl Pts',(17.3764984354523,17.5823449080279,-18.7760619164364));
#90984=CARTESIAN_POINT('Ctrl Pts',(17.4684037333815,17.5099409776383,-18.7686228012944));
#90985=CARTESIAN_POINT('Ctrl Pts',(17.5777443465653,17.4375947898247,-18.7606173499102));
#90986=CARTESIAN_POINT('Ctrl Pts',(17.5897407310793,17.4298307444879,-18.7597493950153));
#90987=CARTESIAN_POINT('Ctrl Pts',(17.6089588054833,17.4176671285735,-18.7583751135059));
#90988=CARTESIAN_POINT('Ctrl Pts',(17.6161296709314,17.4131884393169,-18.7578658590025));
#90989=CARTESIAN_POINT('Ctrl Pts',(17.6288239835789,17.4053653022492,-18.7569704879953));
#90990=CARTESIAN_POINT('Ctrl Pts',(17.6343362262791,17.4020029642941,-18.756583715397));
#90991=CARTESIAN_POINT('Ctrl Pts',(17.6457691779616,17.39510070166,-18.7557856453885));
#90992=CARTESIAN_POINT('Ctrl Pts',(17.6516919855537,17.3915643876897,-18.755374483376));
#90993=CARTESIAN_POINT('Ctrl Pts',(17.6669394831441,17.3825614081306,-18.7543217606395));
#90994=CARTESIAN_POINT('Ctrl Pts',(17.6762890195859,17.3771370500115,-18.7536817412918));
#90995=CARTESIAN_POINT('Ctrl Pts',(17.7154849431519,17.3547960700698,-18.7510209731451));
#90996=CARTESIAN_POINT('Ctrl Pts',(17.7456997529865,17.338534040658,-18.7490237554065));
#90997=CARTESIAN_POINT('Ctrl Pts',(17.8254447535955,17.2980825135208,-18.7438793946618));
#90998=CARTESIAN_POINT('Ctrl Pts',(17.8755486541995,17.2750795785363,-18.7407716463391));
#90999=CARTESIAN_POINT('Ctrl Pts',(18.0275779364744,17.2123469195417,-18.7316269055718));
#91000=CARTESIAN_POINT('Ctrl Pts',(18.1317423635202,17.1785303469814,-18.725738641419));
#91001=CARTESIAN_POINT('Ctrl Pts',(18.2827853535169,17.1421327834214,-18.7172798205953));
#91002=CARTESIAN_POINT('Ctrl Pts',(18.3278564274958,17.1328148848208,-18.7147638427559));
#91003=CARTESIAN_POINT('Ctrl Pts',(18.3949976345574,17.1212019179944,-18.7109848787414));
#91004=CARTESIAN_POINT('Ctrl Pts',(18.4168586877139,17.1177728341217,-18.7097496032274));
#91005=CARTESIAN_POINT('Ctrl Pts',(18.4897488817082,17.1075074530004,-18.7056034016135));
#91006=CARTESIAN_POINT('Ctrl Pts',(18.540969426111,17.1021904362632,-18.7026453026566));
#91007=CARTESIAN_POINT('Ctrl Pts',(18.6009481557041,17.0981675772804,-18.6990774111751));
#91008=CARTESIAN_POINT('Ctrl Pts',(18.6095715108376,17.0976422013584,-18.6985619379131));
#91009=CARTESIAN_POINT('Ctrl Pts',(18.6226567822962,17.0969253487159,-18.6977756241765));
#91010=CARTESIAN_POINT('Ctrl Pts',(18.6271166064366,17.0966951774471,-18.6975069005307));
#91011=CARTESIAN_POINT('Ctrl Pts',(18.6351357887352,17.0963067452077,-18.6970223518697));
#91012=CARTESIAN_POINT('Ctrl Pts',(18.638694844033,17.0961433568516,-18.6968068170462));
#91013=CARTESIAN_POINT('Ctrl Pts',(18.6464438407427,17.095807218253,-18.6963364777056));
#91014=CARTESIAN_POINT('Ctrl Pts',(18.650633834557,17.0956379348362,-18.6960814870096));
#91015=CARTESIAN_POINT('Ctrl Pts',(18.6624421710708,17.0951959942018,-18.6953610274601));
#91016=CARTESIAN_POINT('Ctrl Pts',(18.6700614327788,17.094952039911,-18.6948939986445));
#91017=CARTESIAN_POINT('Ctrl Pts',(18.7164071794245,17.0937186732507,-18.6920407672182));
#91018=CARTESIAN_POINT('Ctrl Pts',(18.755150903648,17.093751331285,-18.6896028560475));
#91019=CARTESIAN_POINT('Ctrl Pts',(18.8845130638409,17.0974111677222,-18.6813339627653));
#91020=CARTESIAN_POINT('Ctrl Pts',(18.9748933270239,17.1057968420952,-18.67534911149));
#91021=CARTESIAN_POINT('Ctrl Pts',(19.1307468895404,17.1304265747517,-18.6649221045853));
#91022=CARTESIAN_POINT('Ctrl Pts',(19.1965088103256,17.1440505528089,-18.6604877009276));
#91023=CARTESIAN_POINT('Ctrl Pts',(19.3726486786,17.1893706001045,-18.6486167278986));
#91024=CARTESIAN_POINT('Ctrl Pts',(19.481287923539,17.2269572220288,-18.6413129003393));
#91025=CARTESIAN_POINT('Ctrl Pts',(19.5994120482589,17.2789145167974,-18.6334336657141));
#91026=CARTESIAN_POINT('Ctrl Pts',(19.6124064104446,17.2847875191501,-18.6325675392087));
#91027=CARTESIAN_POINT('Ctrl Pts',(19.6330013950945,17.2943474954566,-18.6311955965458));
#91028=CARTESIAN_POINT('Ctrl Pts',(19.640640830007,17.2979493628897,-18.6306868679841));
#91029=CARTESIAN_POINT('Ctrl Pts',(19.6540808673365,17.3043847088726,-18.6297921085585));
#91030=CARTESIAN_POINT('Ctrl Pts',(19.6598904095673,17.3071991643812,-18.6294054244209));
#91031=CARTESIAN_POINT('Ctrl Pts',(19.6718843364299,17.313077555936,-18.6286072367332));
#91032=CARTESIAN_POINT('Ctrl Pts',(19.678066800152,17.3161452533802,-18.6281958700613));
#91033=CARTESIAN_POINT('Ctrl Pts',(19.6939073006405,17.324101976521,-18.6271420010573));
#91034=CARTESIAN_POINT('Ctrl Pts',(19.7035431164003,17.3290349820306,-18.6265010466964));
#91035=CARTESIAN_POINT('Ctrl Pts',(19.7436812177253,17.3499735686956,-18.623831174993));
#91036=CARTESIAN_POINT('Ctrl Pts',(19.7738294074527,17.3666490188161,-18.6218259947229));
#91037=CARTESIAN_POINT('Ctrl Pts',(19.8513829707901,17.4120515948756,-18.6166564679669));
#91038=CARTESIAN_POINT('Ctrl Pts',(19.8980917604375,17.4419180076304,-18.6135320235719));
#91039=CARTESIAN_POINT('Ctrl Pts',(20.0335299735626,17.5362092235255,-18.6043581671796));
#91040=CARTESIAN_POINT('Ctrl Pts',(20.1184856894494,17.605726650619,-18.5984573831293));
#91041=CARTESIAN_POINT('Ctrl Pts',(20.2426990019465,17.724595024294,-18.5890955501464));
#91042=CARTESIAN_POINT('Ctrl Pts',(20.2857954782948,17.7696456064384,-18.5856824922175));
#91043=CARTESIAN_POINT('Ctrl Pts',(20.3639009019544,17.8588618271416,-18.5790298687353));
#91044=CARTESIAN_POINT('Ctrl Pts',(20.3992560780308,17.9026515729959,-18.575808071606));
#91045=CARTESIAN_POINT('Ctrl Pts',(20.4380924508417,17.9548806059924,-18.5719465658339));
#91046=CARTESIAN_POINT('Ctrl Pts',(20.4433182616942,17.962001166088,-18.5714197209636));
#91047=CARTESIAN_POINT('Ctrl Pts',(20.4511432900531,17.9728044429518,-18.570619458093));
#91048=CARTESIAN_POINT('Ctrl Pts',(20.4537756290325,17.9764632038733,-18.5703482711729));
#91049=CARTESIAN_POINT('Ctrl Pts',(20.4584693839771,17.9830313287334,-18.5698611007104));
#91050=CARTESIAN_POINT('Ctrl Pts',(20.4605351512207,17.9859375178354,-18.5696454213967));
#91051=CARTESIAN_POINT('Ctrl Pts',(20.4649961534025,17.9922470977984,-18.5691768874961));
#91052=CARTESIAN_POINT('Ctrl Pts',(20.4673886651485,17.9956522906735,-18.5689238582866));
#91053=CARTESIAN_POINT('Ctrl Pts',(20.4740515898102,18.0051951350547,-18.5682143419966));
#91054=CARTESIAN_POINT('Ctrl Pts',(20.4782995001,18.0113483182008,-18.5677563683124));
#91055=CARTESIAN_POINT('Ctrl Pts',(20.5029285736885,18.047431396272,-18.5650685681975));
#91056=CARTESIAN_POINT('Ctrl Pts',(20.522570426062,18.0778558510498,-18.5627936143927));
#91057=CARTESIAN_POINT('Ctrl Pts',(20.583496333549,18.1777609938561,-18.5553330598593));
#91058=CARTESIAN_POINT('Ctrl Pts',(20.6215838303243,18.2491033956708,-18.5500225781887));
#91059=CARTESIAN_POINT('Ctrl Pts',(20.7329514957758,18.4899350182144,-18.5325029595728));
#91060=CARTESIAN_POINT('Ctrl Pts',(20.7881899597197,18.6668744858624,-18.5203483062317));
#91061=CARTESIAN_POINT('Ctrl Pts',(20.8235784259158,18.8706410055578,-18.507628182563));
#91062=CARTESIAN_POINT('Ctrl Pts',(20.8270341684287,18.8925816086989,-18.5062730814037));
#91063=CARTESIAN_POINT('Ctrl Pts',(20.8313307834177,18.9229645714145,-18.5044159762503));
#91064=CARTESIAN_POINT('Ctrl Pts',(20.8324670642412,18.9313630804871,-18.5039046706352));
#91065=CARTESIAN_POINT('Ctrl Pts',(20.8343321484691,18.9458003411262,-18.5030291602133));
#91066=CARTESIAN_POINT('Ctrl Pts',(20.8350854099578,18.951835777502,-18.5026641865368));
#91067=CARTESIAN_POINT('Ctrl Pts',(20.8365834896951,18.9642749905758,-18.5019140543185));
#91068=CARTESIAN_POINT('Ctrl Pts',(20.8373250881334,18.9706790969109,-18.50152900107));
#91069=CARTESIAN_POINT('Ctrl Pts',(20.8389809017083,18.9855730402773,-18.5006360881155));
#91070=CARTESIAN_POINT('Ctrl Pts',(20.8398730331237,18.9940652578583,-18.5001289291483));
#91071=CARTESIAN_POINT('Ctrl Pts',(20.8425572315496,19.0211949452107,-18.4985148279229));
#91072=CARTESIAN_POINT('Ctrl Pts',(20.8441534739472,19.0398512130638,-18.4974140417935));
#91073=CARTESIAN_POINT('Ctrl Pts',(20.8472975665005,19.083391662572,-18.4948648992895));
#91074=CARTESIAN_POINT('Ctrl Pts',(20.8486537855435,19.1082871331505,-18.4934224851758));
#91075=CARTESIAN_POINT('Ctrl Pts',(20.8518757160796,19.1959009129661,-18.4883928072077));
#91076=CARTESIAN_POINT('Ctrl Pts',(20.8513931000354,19.2586747564463,-18.4848740335015));
#91077=CARTESIAN_POINT('Ctrl Pts',(20.8428731269474,19.4219205109642,-18.4758368461326));
#91078=CARTESIAN_POINT('Ctrl Pts',(20.8304524778499,19.5219996806492,-18.4704131036395));
#91079=CARTESIAN_POINT('Ctrl Pts',(20.7965173619992,19.6939835194408,-18.4608625762637));
#91080=CARTESIAN_POINT('Ctrl Pts',(20.7782248413561,19.7663325714297,-18.4567690575104));
#91081=CARTESIAN_POINT('Ctrl Pts',(20.7435199126226,19.8783389424115,-18.4501111135294));
#91082=CARTESIAN_POINT('Ctrl Pts',(20.7296550730301,19.9187229813976,-18.4476423442679));
#91083=CARTESIAN_POINT('Ctrl Pts',(20.7119408020859,19.9656489483421,-18.4446626154238));
#91084=CARTESIAN_POINT('Ctrl Pts',(20.7092644717072,19.9726266243162,-18.4442166127946));
#91085=CARTESIAN_POINT('Ctrl Pts',(20.7048766172369,19.9838878553132,-18.4434918385372));
#91086=CARTESIAN_POINT('Ctrl Pts',(20.7031879132138,19.9881803129204,-18.4432144014202));
#91087=CARTESIAN_POINT('Ctrl Pts',(20.7001655341565,19.9957896998859,-18.4427204347069));
#91088=CARTESIAN_POINT('Ctrl Pts',(20.6988374718782,19.9991088057131,-18.4425042448034));
#91089=CARTESIAN_POINT('Ctrl Pts',(20.6959721824199,20.0062175041717,-18.44203963896));
#91090=CARTESIAN_POINT('Ctrl Pts',(20.6944324032671,20.0100059543564,-18.4417910751516));
#91091=CARTESIAN_POINT('Ctrl Pts',(20.6901712154596,20.020403647306,-18.4411062777548));
#91092=CARTESIAN_POINT('Ctrl Pts',(20.6874273255032,20.0270035349698,-18.4406687174152));
#91093=CARTESIAN_POINT('Ctrl Pts',(20.6725294157162,20.0623317475899,-18.4383114919446));
#91094=CARTESIAN_POINT('Ctrl Pts',(20.6597756524679,20.0908010782994,-18.4363584675208));
#91095=CARTESIAN_POINT('Ctrl Pts',(20.5761200194105,20.266998272962,-18.4239802077525));
#91096=CARTESIAN_POINT('Ctrl Pts',(20.4888965915849,20.4063561070953,-18.4129429647892));
#91097=CARTESIAN_POINT('Ctrl Pts',(20.3132404425781,20.6257141076328,-18.3945844643212));
#91098=CARTESIAN_POINT('Ctrl Pts',(20.2325308660873,20.7109431651765,-18.3871201421978));
#91099=CARTESIAN_POINT('Ctrl Pts',(20.1345138028437,20.7985939041118,-18.379091234928));
#91100=CARTESIAN_POINT('Ctrl Pts',(20.1237623200426,20.808014096948,-18.3782229768817));
#91101=CARTESIAN_POINT('Ctrl Pts',(20.1064999679573,20.8228326027197,-18.3768483076294));
#91102=CARTESIAN_POINT('Ctrl Pts',(20.1000508823782,20.8283019171533,-18.3763389659636));
#91103=CARTESIAN_POINT('Ctrl Pts',(20.0886197264919,20.8378792483207,-18.3754434935676));
#91104=CARTESIAN_POINT('Ctrl Pts',(20.0836513391528,20.8420033587254,-18.3750567062754));
#91105=CARTESIAN_POINT('Ctrl Pts',(20.073336690675,20.8504858354867,-18.3742586555995));
#91106=CARTESIAN_POINT('Ctrl Pts',(20.0679878359118,20.8548409385097,-18.3738475273687));
#91107=CARTESIAN_POINT('Ctrl Pts',(20.054204685956,20.8659517699852,-18.3727949938832));
#91108=CARTESIAN_POINT('Ctrl Pts',(20.0457397103835,20.8726692548624,-18.3721551289169));
#91109=CARTESIAN_POINT('Ctrl Pts',(20.0102059305757,20.9004267658756,-18.3694958609134));
#91110=CARTESIAN_POINT('Ctrl Pts',(19.9826785877602,20.9208731985757,-18.3674999550833));
#91111=CARTESIAN_POINT('Ctrl Pts',(19.9096820194307,20.9723892641537,-18.3623597366743));
#91112=CARTESIAN_POINT('Ctrl Pts',(19.8634751073856,21.0023701394384,-18.359254735634));
#91113=CARTESIAN_POINT('Ctrl Pts',(19.7278399868876,21.0830384852254,-18.3504795520042));
#91114=CARTESIAN_POINT('Ctrl Pts',(19.6358217887229,21.129062674551,-18.3449342414303));
#91115=CARTESIAN_POINT('Ctrl Pts',(19.4803921384489,21.193135339703,-18.3357919712046));
#91116=CARTESIAN_POINT('Ctrl Pts',(19.4188406381593,21.2152340843411,-18.3322230005182));
#91117=CARTESIAN_POINT('Ctrl Pts',(19.2986467218889,21.2522031027207,-18.3251903183212));
#91118=CARTESIAN_POINT('Ctrl Pts',(19.2401969974864,21.2674773773786,-18.3217422066224));
#91119=CARTESIAN_POINT('Ctrl Pts',(19.1724050180915,21.2821278683357,-18.3176284693294));
#91120=CARTESIAN_POINT('Ctrl Pts',(19.1636176693573,21.283968465418,-18.3170930492486));
#91121=CARTESIAN_POINT('Ctrl Pts',(19.1503712301684,21.2866552208166,-18.3162822813292));
#91122=CARTESIAN_POINT('Ctrl Pts',(19.1459205631155,21.287543051761,-18.3160092525769));
#91123=CARTESIAN_POINT('Ctrl Pts',(19.137965754997,21.2891033179351,-18.3155200996695));
#91124=CARTESIAN_POINT('Ctrl Pts',(19.1344627376407,21.2897812118468,-18.3153042902113));
#91125=CARTESIAN_POINT('Ctrl Pts',(19.1268921650512,21.291226401109,-18.3148370061301));
#91126=CARTESIAN_POINT('Ctrl Pts',(19.1228241255658,21.2919906131287,-18.3145853651313));
#91127=CARTESIAN_POINT('Ctrl Pts',(19.1115024688403,21.2940831153999,-18.3138835608291));
#91128=CARTESIAN_POINT('Ctrl Pts',(19.1042441950608,21.2953854278869,-18.3134319616598));
#91129=CARTESIAN_POINT('Ctrl Pts',(19.0640941151047,21.3023730111874,-18.3109251948959));
#91130=CARTESIAN_POINT('Ctrl Pts',(19.0310801517453,21.3073173164746,-18.308831837261));
#91131=CARTESIAN_POINT('Ctrl Pts',(18.8373274374331,21.3316660523057,-18.2964121022734));
#91132=CARTESIAN_POINT('Ctrl Pts',(18.6749084259211,21.3333593728565,-18.2855110039595));
#91133=CARTESIAN_POINT('Ctrl Pts',(18.3979808907166,21.3044088446963,-18.2673255427473));
#91134=CARTESIAN_POINT('Ctrl Pts',(18.2832615100843,21.2827412966339,-18.2599031283738));
#91135=CARTESIAN_POINT('Ctrl Pts',(18.1571215317626,21.247935028918,-18.2519132285541));
#91136=CARTESIAN_POINT('Ctrl Pts',(18.1433891043865,21.24399578574,-18.2510454814046));
#91137=CARTESIAN_POINT('Ctrl Pts',(18.1215956219463,21.2375047096665,-18.2496714656165));
#91138=CARTESIAN_POINT('Ctrl Pts',(18.1135083461791,21.2350431248708,-18.2491622708503));
#91139=CARTESIAN_POINT('Ctrl Pts',(18.0992705579791,21.2306161076688,-18.2482669693244));
#91140=CARTESIAN_POINT('Ctrl Pts',(18.0931139268971,21.228670867525,-18.2478802067905));
#91141=CARTESIAN_POINT('Ctrl Pts',(18.0803978493686,21.2245890389854,-18.2470821235026));
#91142=CARTESIAN_POINT('Ctrl Pts',(18.0738397470212,21.2224484908521,-18.2466709383143));
#91143=CARTESIAN_POINT('Ctrl Pts',(18.0570316228513,21.2168713035411,-18.2456180857522));
#91144=CARTESIAN_POINT('Ctrl Pts',(18.046797169997,21.2133881109883,-18.2449779605012));
#91145=CARTESIAN_POINT('Ctrl Pts',(18.0047966138133,21.1987337032221,-18.2423544822049));
#91146=CARTESIAN_POINT('Ctrl Pts',(17.973271515087,21.1868834003443,-18.2403936947547));
#91147=CARTESIAN_POINT('Ctrl Pts',(17.8919727815959,21.1540887572778,-18.2353480330195));
#91148=CARTESIAN_POINT('Ctrl Pts',(17.8426930477131,21.1319831557131,-18.2323009089659));
#91149=CARTESIAN_POINT('Ctrl Pts',(17.6803078053599,21.0515453373463,-18.2222154748355));
#91150=CARTESIAN_POINT('Ctrl Pts',(17.5716302879619,20.9849141487426,-18.2154056689656));
#91151=CARTESIAN_POINT('Ctrl Pts',(17.3877165111387,20.8479577562523,-18.2028664177071));
#91152=CARTESIAN_POINT('Ctrl Pts',(17.3103691858698,20.7811527490037,-18.1971988929064));
#91153=CARTESIAN_POINT('Ctrl Pts',(17.2312944836335,20.7021938329868,-18.1905785134173));
#91154=CARTESIAN_POINT('Ctrl Pts',(17.2244841048952,20.6952993871924,-18.1900010124083));
#91155=CARTESIAN_POINT('Ctrl Pts',(17.2144982268534,20.6850504381913,-18.1891429160332));
#91156=CARTESIAN_POINT('Ctrl Pts',(17.2112858742539,20.6817317985459,-18.1888651213047));
#91157=CARTESIAN_POINT('Ctrl Pts',(17.205605977836,20.6758254156188,-18.1883707601584));
#91158=CARTESIAN_POINT('Ctrl Pts',(17.2031341027575,20.6732419053222,-18.188154535459));
#91159=CARTESIAN_POINT('Ctrl Pts',(17.1978517444917,20.6676929084314,-18.1876901289652));
#91160=CARTESIAN_POINT('Ctrl Pts',(17.1950433396301,20.6647255893828,-18.1874418007334));
#91161=CARTESIAN_POINT('Ctrl Pts',(17.1892976819905,20.6586195039357,-18.1869308575326));
#91162=CARTESIAN_POINT('Ctrl Pts',(17.1863613663141,20.6554798850187,-18.186668174419));
#91163=CARTESIAN_POINT('Ctrl Pts',(17.172907708721,20.641006617132,-18.1854574802763));
#91164=CARTESIAN_POINT('Ctrl Pts',(17.1625054852299,20.6295672437599,-18.1845012580124));
#91165=CARTESIAN_POINT('Ctrl Pts',(17.0941974973345,20.5527752339454,-18.1780928157282));
#91166=CARTESIAN_POINT('Ctrl Pts',(17.0402626618156,20.4840136367756,-18.1724082045646));
#91167=CARTESIAN_POINT('Ctrl Pts',(16.9494514375479,20.3522138990728,-18.161872553892));
#91168=CARTESIAN_POINT('Ctrl Pts',(16.9112865550028,20.2902120188646,-18.157046711364));
#91169=CARTESIAN_POINT('Ctrl Pts',(16.8741069813084,20.2221921702089,-18.1519487845772));
#91170=CARTESIAN_POINT('Ctrl Pts',(16.8718386237847,20.2180087662163,-18.1516360039948));
#91171=CARTESIAN_POINT('Ctrl Pts',(16.8058494071645,20.0953231363686,-18.1424856013833));
#91172=CARTESIAN_POINT('Ctrl Pts',(16.7535466359384,19.9710054393493,-18.133855260602));
#91173=CARTESIAN_POINT('Ctrl Pts',(16.708693751212,19.8274997919292,-18.1246738677132));
#91174=CARTESIAN_POINT('Ctrl Pts',(16.7041601068514,19.8124045427961,-18.123716947619));
#91175=CARTESIAN_POINT('Ctrl Pts',(16.697560032873,19.7895035996151,-18.1222782772424));
#91176=CARTESIAN_POINT('Ctrl Pts',(16.6953690586117,19.7817346512263,-18.121792479011));
#91177=CARTESIAN_POINT('Ctrl Pts',(16.6915244699324,19.7677975267565,-18.1209249599746));
#91178=CARTESIAN_POINT('Ctrl Pts',(16.6898542383331,19.7616340737468,-18.1205427029385));
#91179=CARTESIAN_POINT('Ctrl Pts',(16.6863713131476,19.7485471872113,-18.1197339567774));
#91180=CARTESIAN_POINT('Ctrl Pts',(16.6845657850353,19.7416219163989,-18.119307704042));
#91181=CARTESIAN_POINT('Ctrl Pts',(16.6809624106151,19.7275080461815,-18.1184424219227));
#91182=CARTESIAN_POINT('Ctrl Pts',(16.6791671181765,19.7203188933179,-18.1180034797745));
#91183=CARTESIAN_POINT('Ctrl Pts',(16.6747876919973,19.7023815898169,-18.1169127010839));
#91184=CARTESIAN_POINT('Ctrl Pts',(16.6722499088747,19.6916222683857,-18.1162623493033));
#91185=CARTESIAN_POINT('Ctrl Pts',(16.6345655716973,19.5260604238103,-18.1063131420913));
#91186=CARTESIAN_POINT('Ctrl Pts',(16.6168549651969,19.3678091385423,-18.0976369978758));
#91187=CARTESIAN_POINT('Ctrl Pts',(16.6170008943746,19.2090540346034,-18.089014728333));
#91188=CARTESIAN_POINT('Ctrl Pts',(16.6170008942678,19.2090541508675,-18.0890147346475));
#91189=CARTESIAN_POINT('Ctrl Pts',(16.6171322447143,19.0661505859132,-18.0812533901164));
#91190=CARTESIAN_POINT('Ctrl Pts',(16.6317328296694,18.9236421400003,-18.0735575474113));
#91191=CARTESIAN_POINT('Ctrl Pts',(16.66253979312,18.7741512307517,-18.0645864550536));
#91192=CARTESIAN_POINT('Ctrl Pts',(16.6645755328753,18.7646071203777,-18.0640096344675));
#91193=CARTESIAN_POINT('Ctrl Pts',(16.6678825024972,18.7496120812857,-18.0630964765093));
#91194=CARTESIAN_POINT('Ctrl Pts',(16.6691095143436,18.7441514103039,-18.0627624919851));
#91195=CARTESIAN_POINT('Ctrl Pts',(16.6714748390661,18.7338165827897,-18.0621275467242));
#91196=CARTESIAN_POINT('Ctrl Pts',(16.672608815234,18.7289414606676,-18.0618268279476));
#91197=CARTESIAN_POINT('Ctrl Pts',(16.6745951113992,18.7205372740482,-18.0613062705801));
#91198=CARTESIAN_POINT('Ctrl Pts',(16.6754392490442,18.7170062599395,-18.0610869016675));
#91199=CARTESIAN_POINT('Ctrl Pts',(16.6770954354609,18.7101564253846,-18.0606600439741));
#91200=CARTESIAN_POINT('Ctrl Pts',(16.6779064370994,18.7068373932249,-18.060452621718));
#91201=CARTESIAN_POINT('Ctrl Pts',(16.6801203219178,18.6978712381477,-18.0598907105575));
#91202=CARTESIAN_POINT('Ctrl Pts',(16.6815384465943,18.692227961207,-18.0595353560513));
#91203=CARTESIAN_POINT('Ctrl Pts',(16.6869129238201,18.6712078135313,-18.0582056095516));
#91204=CARTESIAN_POINT('Ctrl Pts',(16.6910188512614,18.6558702012061,-18.0572231157216));
#91205=CARTESIAN_POINT('Ctrl Pts',(16.7100001833739,18.5880300928202,-18.0528274467239));
#91206=CARTESIAN_POINT('Ctrl Pts',(16.7267222361259,18.5360951484225,-18.0493292904414));
#91207=CARTESIAN_POINT('Ctrl Pts',(16.7454193875989,18.4848897136231,-18.0457833433865));
#91208=CARTESIAN_POINT('Origin',(18.734,19.211,0.));
#91209=CARTESIAN_POINT('',(16.7454194502294,18.4848895420984,-17.2426989706651));
#91210=CARTESIAN_POINT('',(16.7454194505834,18.4848895411289,-17.4677764891862));
#91211=CARTESIAN_POINT('',(16.7454194503191,18.4848895418526,0.));
#91212=CARTESIAN_POINT('Ctrl Pts',(16.7454194505834,18.4848895411289,-17.4677764891862));
#91213=CARTESIAN_POINT('Ctrl Pts',(16.7278145381498,18.5331036744084,-17.471069432283));
#91214=CARTESIAN_POINT('Ctrl Pts',(16.7119674259087,18.5819461488812,-17.4743159633458));
#91215=CARTESIAN_POINT('Ctrl Pts',(16.6884846851829,18.6644279468596,-17.4796471179921));
#91216=CARTESIAN_POINT('Ctrl Pts',(16.6798675453392,18.6977612741547,-17.4817614577792));
#91217=CARTESIAN_POINT('Ctrl Pts',(16.6696144590733,18.741832165455,-17.4845061250789));
#91218=CARTESIAN_POINT('Ctrl Pts',(16.6672430098837,18.7523915949572,-17.485159967894));
#91219=CARTESIAN_POINT('Ctrl Pts',(16.6634921057334,18.7697136033824,-17.4862264849215));
#91220=CARTESIAN_POINT('Ctrl Pts',(16.6620645844282,18.7764654679844,-17.486640694217));
#91221=CARTESIAN_POINT('Ctrl Pts',(16.6593656416378,18.7895466182744,-17.4874403240723));
#91222=CARTESIAN_POINT('Ctrl Pts',(16.6580901071216,18.7958749683059,-17.4878258722433));
#91223=CARTESIAN_POINT('Ctrl Pts',(16.6552123719551,18.8104973739121,-17.4887137889343));
#91224=CARTESIAN_POINT('Ctrl Pts',(16.6536308200333,18.8187954179053,-17.4892154938139));
#91225=CARTESIAN_POINT('Ctrl Pts',(16.6495122698741,18.8411305999054,-17.4905601779181));
#91226=CARTESIAN_POINT('Ctrl Pts',(16.6470673782895,18.8551844333864,-17.4914002290407));
#91227=CARTESIAN_POINT('Ctrl Pts',(16.6261906875318,18.9828153699925,-17.4989768923311));
#91228=CARTESIAN_POINT('Ctrl Pts',(16.6169037092498,19.0977007839662,-17.5054070942451));
#91229=CARTESIAN_POINT('Ctrl Pts',(16.6171578063362,19.3990360603433,-17.5219135172291));
#91230=CARTESIAN_POINT('Ctrl Pts',(16.6418924522489,19.5844189884413,-17.5316811019748));
#91231=CARTESIAN_POINT('Ctrl Pts',(16.6942562458898,19.7778655756035,-17.5434580591134));
#91232=CARTESIAN_POINT('Ctrl Pts',(16.6981093688598,19.7915518726192,-17.5443004486877));
#91233=CARTESIAN_POINT('Ctrl Pts',(16.7036607297278,19.810535127945,-17.5454829879046));
#91234=CARTESIAN_POINT('Ctrl Pts',(16.7052425223367,19.8158661151707,-17.5458166329892));
#91235=CARTESIAN_POINT('Ctrl Pts',(16.70781564287,19.8244144478422,-17.5463542340038));
#91236=CARTESIAN_POINT('Ctrl Pts',(16.7087936869134,19.8276358106429,-17.546557417383));
#91237=CARTESIAN_POINT('Ctrl Pts',(16.7108530777658,19.8343610330275,-17.5469828690383));
#91238=CARTESIAN_POINT('Ctrl Pts',(16.7119358448849,19.8378644178034,-17.5472052228027));
#91239=CARTESIAN_POINT('Ctrl Pts',(16.7145777282274,19.8463343894496,-17.5477445178966));
#91240=CARTESIAN_POINT('Ctrl Pts',(16.7161460667055,19.8512980561515,-17.5480619953759));
#91241=CARTESIAN_POINT('Ctrl Pts',(16.7216994325126,19.868650971913,-17.5491767913443));
#91242=CARTESIAN_POINT('Ctrl Pts',(16.7257802914508,19.8810089235115,-17.5499794559409));
#91243=CARTESIAN_POINT('Ctrl Pts',(16.750571251162,19.9538209765807,-17.5547573412506));
#91244=CARTESIAN_POINT('Ctrl Pts',(16.7738944100975,20.0133447680255,-17.5588615547738));
#91245=CARTESIAN_POINT('Ctrl Pts',(16.8760923080288,20.2429951840857,-17.5752528654356));
#91246=CARTESIAN_POINT('Ctrl Pts',(16.974746264155,20.4034264307322,-17.5878515501128));
#91247=CARTESIAN_POINT('Ctrl Pts',(17.1286546429515,20.5921933516103,-17.6032548845364));
#91248=CARTESIAN_POINT('Ctrl Pts',(17.1657758433198,20.6342015705637,-17.6067354194405));
#91249=CARTESIAN_POINT('Ctrl Pts',(17.2128425227556,20.6833836833239,-17.6108793252361));
#91250=CARTESIAN_POINT('Ctrl Pts',(17.2212358818161,20.692005912753,-17.611608560134));
#91251=CARTESIAN_POINT('Ctrl Pts',(17.2352366845433,20.7061452736404,-17.6128091588313));
#91252=CARTESIAN_POINT('Ctrl Pts',(17.2408020960839,20.7117034641773,-17.6132823519281));
#91253=CARTESIAN_POINT('Ctrl Pts',(17.2509287741856,20.7217048960451,-17.614136123977));
#91254=CARTESIAN_POINT('Ctrl Pts',(17.2554793349983,20.7261587996999,-17.6145171714241));
#91255=CARTESIAN_POINT('Ctrl Pts',(17.2652853757592,20.7356703085867,-17.6153327649525));
#91256=CARTESIAN_POINT('Ctrl Pts',(17.2705470492769,20.7407214322899,-17.6157670254912));
#91257=CARTESIAN_POINT('Ctrl Pts',(17.2849677660904,20.7544225901594,-17.616948154851));
#91258=CARTESIAN_POINT('Ctrl Pts',(17.2941781765849,20.7630183097727,-17.6176926787737));
#91259=CARTESIAN_POINT('Ctrl Pts',(17.3433135806804,20.8080606057894,-17.6216137775313));
#91260=CARTESIAN_POINT('Ctrl Pts',(17.3845489113014,20.8430520145755,-17.6247285072309));
#91261=CARTESIAN_POINT('Ctrl Pts',(17.5775460280295,20.9945034180545,-17.6386250069292));
#91262=CARTESIAN_POINT('Ctrl Pts',(17.7433022263399,21.0916335286676,-17.6486492253669));
#91263=CARTESIAN_POINT('Ctrl Pts',(17.9351125746571,21.1715462468961,-17.6602003078369));
#91264=CARTESIAN_POINT('Ctrl Pts',(17.950457994147,21.1777294195228,-17.6611247770083));
#91265=CARTESIAN_POINT('Ctrl Pts',(18.0154375139924,21.2030306048585,-17.6650468978339));
#91266=CARTESIAN_POINT('Ctrl Pts',(18.0657063777173,21.2204528111761,-17.6680992472002));
#91267=CARTESIAN_POINT('Ctrl Pts',(18.1249049324642,21.2385029156948,-17.6717720071343));
#91268=CARTESIAN_POINT('Ctrl Pts',(18.1332522675775,21.2409918794265,-17.6722916723895));
#91269=CARTESIAN_POINT('Ctrl Pts',(18.1459167026367,21.2446831405404,-17.6730831307443));
#91270=CARTESIAN_POINT('Ctrl Pts',(18.1502227682919,21.2459233950315,-17.6733527652239));
#91271=CARTESIAN_POINT('Ctrl Pts',(18.1579604287672,21.24812545351,-17.6738382792656));
#91272=CARTESIAN_POINT('Ctrl Pts',(18.1613905405095,21.2490922716031,-17.6740538634403));
#91273=CARTESIAN_POINT('Ctrl Pts',(18.1688506234465,21.2511746657762,-17.6745235166991));
#91274=CARTESIAN_POINT('Ctrl Pts',(18.1728814107155,21.2522869501261,-17.674777767616));
#91275=CARTESIAN_POINT('Ctrl Pts',(18.1842167233877,21.2553787867753,-17.6754940931238));
#91276=CARTESIAN_POINT('Ctrl Pts',(18.191528521107,21.2573310987412,-17.6759576997751));
#91277=CARTESIAN_POINT('Ctrl Pts',(18.2353830048929,21.2687890615176,-17.6787468828349));
#91278=CARTESIAN_POINT('Ctrl Pts',(18.2721618032511,21.2773542294488,-17.6811215649766));
#91279=CARTESIAN_POINT('Ctrl Pts',(18.3941309889349,21.3023400940216,-17.6890700032577));
#91280=CARTESIAN_POINT('Ctrl Pts',(18.4800992851541,21.3145082245148,-17.6947858486727));
#91281=CARTESIAN_POINT('Ctrl Pts',(18.741827592304,21.3352735164521,-17.7121325352482));
#91282=CARTESIAN_POINT('Ctrl Pts',(18.9181763674323,21.3272943791837,-17.7236768236546));
#91283=CARTESIAN_POINT('Ctrl Pts',(19.1141646073011,21.2937124697931,-17.7359157476735));
#91284=CARTESIAN_POINT('Ctrl Pts',(19.1367351307694,21.2894659824281,-17.7373176168934));
#91285=CARTESIAN_POINT('Ctrl Pts',(19.1685800735477,21.2829363417795,-17.7392854326175));
#91286=CARTESIAN_POINT('Ctrl Pts',(19.1779143889847,21.2809565368931,-17.7398610030083));
#91287=CARTESIAN_POINT('Ctrl Pts',(19.1930627928452,21.2776363844247,-17.7407931594251));
#91288=CARTESIAN_POINT('Ctrl Pts',(19.1988850849014,21.2763344649648,-17.741150971393));
#91289=CARTESIAN_POINT('Ctrl Pts',(19.211063708426,21.2735571013614,-17.7418984756122));
#91290=CARTESIAN_POINT('Ctrl Pts',(19.2174188868234,21.272076844663,-17.7422880089456));
#91291=CARTESIAN_POINT('Ctrl Pts',(19.232526428858,21.2684842558276,-17.7432127775852));
#91292=CARTESIAN_POINT('Ctrl Pts',(19.2412724063549,21.2663454144774,-17.743747153775));
#91293=CARTESIAN_POINT('Ctrl Pts',(19.2707149375798,21.2589458212547,-17.7455429570136));
#91294=CARTESIAN_POINT('Ctrl Pts',(19.2913458872534,21.2534276295855,-17.7467960732497));
#91295=CARTESIAN_POINT('Ctrl Pts',(19.4033557192912,21.2216445272356,-17.753576137664));
#91296=CARTESIAN_POINT('Ctrl Pts',(19.492974382584,21.1895574117104,-17.7589087810605));
#91297=CARTESIAN_POINT('Ctrl Pts',(19.7363095986762,21.0834556104271,-17.7735133182203));
#91298=CARTESIAN_POINT('Ctrl Pts',(19.8836685566068,20.9967672952764,-17.7824758109733));
#91299=CARTESIAN_POINT('Ctrl Pts',(20.0485503306469,20.8708271237563,-17.7943218991438));
#91300=CARTESIAN_POINT('Ctrl Pts',(20.0774678139186,20.8475092448898,-17.7964788729866));
#91301=CARTESIAN_POINT('Ctrl Pts',(20.1112112788538,20.8188026655144,-17.7991125988913));
#91302=CARTESIAN_POINT('Ctrl Pts',(20.1166438930873,20.8141332382076,-17.7995403465985));
#91303=CARTESIAN_POINT('Ctrl Pts',(20.1254646639922,20.8064734438604,-17.8002411667417));
#91304=CARTESIAN_POINT('Ctrl Pts',(20.1288671799788,20.8034995982892,-17.8005130443811));
#91305=CARTESIAN_POINT('Ctrl Pts',(20.1349379838007,20.7981592502612,-17.8010009562064));
#91306=CARTESIAN_POINT('Ctrl Pts',(20.1376098358062,20.7957968793201,-17.8012166822356));
#91307=CARTESIAN_POINT('Ctrl Pts',(20.1433801608473,20.7906688927959,-17.8016847379081));
#91308=CARTESIAN_POINT('Ctrl Pts',(20.1464764263562,20.7879009458304,-17.8019372390437));
#91309=CARTESIAN_POINT('Ctrl Pts',(20.1550950819255,20.780150436122,-17.8026438184658));
#91310=CARTESIAN_POINT('Ctrl Pts',(20.160599324441,20.7751479107757,-17.8030993639404));
#91311=CARTESIAN_POINT('Ctrl Pts',(20.1922708963681,20.7460569945044,-17.8057449268417));
#91312=CARTESIAN_POINT('Ctrl Pts',(20.2178525815749,20.7213427274424,-17.8079784654129));
#91313=CARTESIAN_POINT('Ctrl Pts',(20.2978171774206,20.6400965326136,-17.8152423233763));
#91314=CARTESIAN_POINT('Ctrl Pts',(20.3496837032355,20.5811845037461,-17.8203908452554));
#91315=CARTESIAN_POINT('Ctrl Pts',(20.514464659045,20.3716207401282,-17.8379867275695));
#91316=CARTESIAN_POINT('Ctrl Pts',(20.6105582562123,20.2088240356525,-17.8503962460361));
#91317=CARTESIAN_POINT('Ctrl Pts',(20.6923702539724,20.015333087509,-17.8633119731376));
#91318=CARTESIAN_POINT('Ctrl Pts',(20.7005622604193,19.9950910018949,-17.8646439180138));
#91319=CARTESIAN_POINT('Ctrl Pts',(20.7114759711671,19.9668760547626,-17.8664746012221));
#91320=CARTESIAN_POINT('Ctrl Pts',(20.7144652639641,19.9590088021795,-17.8669823003044));
#91321=CARTESIAN_POINT('Ctrl Pts',(20.7195285507188,19.9454400440436,-17.8678532649114));
#91322=CARTESIAN_POINT('Ctrl Pts',(20.7216250794035,19.9397471090383,-17.8682172814285));
#91323=CARTESIAN_POINT('Ctrl Pts',(20.7259018044506,19.9279782907146,-17.8689669318332));
#91324=CARTESIAN_POINT('Ctrl Pts',(20.7280787429726,19.921901284412,-17.869352453872));
#91325=CARTESIAN_POINT('Ctrl Pts',(20.733088397827,19.9077125658525,-17.8702489681924));
#91326=CARTESIAN_POINT('Ctrl Pts',(20.7358996073823,19.8995933393707,-17.8707592418767));
#91327=CARTESIAN_POINT('Ctrl Pts',(20.7447725785032,19.8734531148339,-17.872393474927));
#91328=CARTESIAN_POINT('Ctrl Pts',(20.7506411364583,19.8553671728449,-17.8735110562459));
#91329=CARTESIAN_POINT('Ctrl Pts',(20.7789116014426,19.7640704598513,-17.8790902698697));
#91330=CARTESIAN_POINT('Ctrl Pts',(20.7975753557142,19.6897577025538,-17.8834287521325));
#91331=CARTESIAN_POINT('Ctrl Pts',(20.8331254686511,19.5067026779437,-17.8937918397514));
#91332=CARTESIAN_POINT('Ctrl Pts',(20.8456447165604,19.397347030519,-17.8997070761613));
#91333=CARTESIAN_POINT('Ctrl Pts',(20.852163677474,19.2170914331259,-17.90953068319));
#91334=CARTESIAN_POINT('Ctrl Pts',(20.8511926986483,19.1465921290349,-17.9133941242643));
#91335=CARTESIAN_POINT('Ctrl Pts',(20.8436648199995,19.0285407420244,-17.9200783564362));
#91336=CARTESIAN_POINT('Ctrl Pts',(20.8390039902355,18.9809250615126,-17.9228339540835));
#91337=CARTESIAN_POINT('Ctrl Pts',(20.8317210118101,18.9258414011549,-17.9261328082676));
#91338=CARTESIAN_POINT('Ctrl Pts',(20.8306647736406,18.9181763453397,-17.9265943689256));
#91339=CARTESIAN_POINT('Ctrl Pts',(20.8289077477013,18.9059228417631,-17.9273365017912));
#91340=CARTESIAN_POINT('Ctrl Pts',(20.82823383626,18.9013305278501,-17.9276155970307));
#91341=CARTESIAN_POINT('Ctrl Pts',(20.8270122832189,18.8931927429871,-17.9281119314208));
#91342=CARTESIAN_POINT('Ctrl Pts',(20.8264707254483,18.8896464045768,-17.9283288240676));
#91343=CARTESIAN_POINT('Ctrl Pts',(20.8253023152921,18.8821233780297,-17.9287902170686));
#91344=CARTESIAN_POINT('Ctrl Pts',(20.8246731432062,18.8781471585274,-17.9290348410504));
#91345=CARTESIAN_POINT('Ctrl Pts',(20.8229412017746,18.8674003599248,-17.9296980122098));
#91346=CARTESIAN_POINT('Ctrl Pts',(20.8218168699204,18.8606333751208,-17.9301177528161));
#91347=CARTESIAN_POINT('Ctrl Pts',(20.8160296030717,18.8268190026475,-17.9322255765431));
#91348=CARTESIAN_POINT('Ctrl Pts',(20.8108741000732,18.7998599839208,-17.9339393555694));
#91349=CARTESIAN_POINT('Ctrl Pts',(20.7943756947817,18.7218411635685,-17.938981270215));
#91350=CARTESIAN_POINT('Ctrl Pts',(20.7816632939064,18.6710938347364,-17.9423637066549));
#91351=CARTESIAN_POINT('Ctrl Pts',(20.7281508699135,18.4867346121005,-17.9549159520242));
#91352=CARTESIAN_POINT('Ctrl Pts',(20.676031861902,18.3567665953127,-17.9642561577558));
#91353=CARTESIAN_POINT('Ctrl Pts',(20.568025803529,18.1494501516391,-17.9793774121036));
#91354=CARTESIAN_POINT('Ctrl Pts',(20.5190441747391,18.0690016554109,-17.9853157197031));
#91355=CARTESIAN_POINT('Ctrl Pts',(20.4569072706104,17.9807680760621,-17.9919011250461));
#91356=CARTESIAN_POINT('Ctrl Pts',(20.4488381347374,17.9695451133157,-17.9927403433996));
#91357=CARTESIAN_POINT('Ctrl Pts',(20.4357377078108,17.9516958399824,-17.9940778131357));
#91358=CARTESIAN_POINT('Ctrl Pts',(20.4307763725365,17.9450189028627,-17.9945787533409));
#91359=CARTESIAN_POINT('Ctrl Pts',(20.4219072802446,17.9332287276212,-17.9954644985758));
#91360=CARTESIAN_POINT('Ctrl Pts',(20.4180153438979,17.9281037710892,-17.9958499152712));
#91361=CARTESIAN_POINT('Ctrl Pts',(20.4098676450413,17.9174757328825,-17.996650060495));
#91362=CARTESIAN_POINT('Ctrl Pts',(20.4056079990364,17.9119757151419,-17.9970646294719));
#91363=CARTESIAN_POINT('Ctrl Pts',(20.3944973180197,17.8977748499481,-17.998136383414));
#91364=CARTESIAN_POINT('Ctrl Pts',(20.3876049277941,17.8891065142371,-17.9987919162296));
#91365=CARTESIAN_POINT('Ctrl Pts',(20.3575847336181,17.8519533257188,-18.0016078413936));
#91366=CARTESIAN_POINT('Ctrl Pts',(20.3337857501951,17.8240172883197,-18.0037410557394));
#91367=CARTESIAN_POINT('Ctrl Pts',(20.2688577207695,17.7516986906226,-18.0093211374301));
#91368=CARTESIAN_POINT('Ctrl Pts',(20.2265311953206,17.7084355318785,-18.0127192631978));
#91369=CARTESIAN_POINT('Ctrl Pts',(20.0626353976562,17.5546827378792,-18.0251630816708));
#91370=CARTESIAN_POINT('Ctrl Pts',(19.9302075613234,17.4566512418382,-18.0338183669568));
#91371=CARTESIAN_POINT('Ctrl Pts',(19.7389938622242,17.3469071906713,-18.0461877225001));
#91372=CARTESIAN_POINT('Ctrl Pts',(19.6891028610983,17.3208592611254,-18.0494095568747));
#91373=CARTESIAN_POINT('Ctrl Pts',(19.6302525253493,17.2930588058304,-18.053271104193));
#91374=CARTESIAN_POINT('Ctrl Pts',(19.6222428771549,17.2893362420735,-18.0537979506305));
#91375=CARTESIAN_POINT('Ctrl Pts',(19.6101110613525,17.2837899117377,-18.054598215452));
#91376=CARTESIAN_POINT('Ctrl Pts',(19.6060058641526,17.2819289572066,-18.05486940274));
#91377=CARTESIAN_POINT('Ctrl Pts',(19.5986425598896,17.2786193549091,-18.0553565736344));
#91378=CARTESIAN_POINT('Ctrl Pts',(19.5953867094193,17.2771658161954,-18.0555722530103));
#91379=CARTESIAN_POINT('Ctrl Pts',(19.5883227022054,17.2740335469633,-18.0560407867821));
#91380=CARTESIAN_POINT('Ctrl Pts',(19.5845133145256,17.2723578409569,-18.056293815799));
#91381=CARTESIAN_POINT('Ctrl Pts',(19.5738460019558,17.2677029047829,-18.0570033308837));
#91382=CARTESIAN_POINT('Ctrl Pts',(19.5669772769126,17.2647487932967,-18.057461303547));
#91383=CARTESIAN_POINT('Ctrl Pts',(19.5267536975942,17.2477013094374,-18.0601490847304));
#91384=CARTESIAN_POINT('Ctrl Pts',(19.4930594299405,17.2344300942969,-18.0624240198908));
#91385=CARTESIAN_POINT('Ctrl Pts',(19.3831204868046,17.1943537867052,-18.0698844847535));
#91386=CARTESIAN_POINT('Ctrl Pts',(19.3056795058767,17.1710489807659,-18.0751948922975));
#91387=CARTESIAN_POINT('Ctrl Pts',(19.047642151826,17.1092457342018,-18.0927145441974));
#91388=CARTESIAN_POINT('Ctrl Pts',(18.8632910545939,17.089902785717,-18.1048693120295));
#91389=CARTESIAN_POINT('Ctrl Pts',(18.6565433610784,17.0953008944633,-18.1175895244022));
#91390=CARTESIAN_POINT('Ctrl Pts',(18.6343518742613,17.0962299070359,-18.1189446157085));
#91391=CARTESIAN_POINT('Ctrl Pts',(18.6037176416392,17.0979956625955,-18.1208017097063));
#91392=CARTESIAN_POINT('Ctrl Pts',(18.5952597625058,17.098534148783,-18.121313013871));
#91393=CARTESIAN_POINT('Ctrl Pts',(18.5807377890449,17.0995463093912,-18.1221885225074));
#91394=CARTESIAN_POINT('Ctrl Pts',(18.5746721325546,17.0999953517938,-18.1225534958415));
#91395=CARTESIAN_POINT('Ctrl Pts',(18.5621813314149,17.1009741929067,-18.1233036279888));
#91396=CARTESIAN_POINT('Ctrl Pts',(18.5557564971343,17.1015072134328,-18.1236886815058));
#91397=CARTESIAN_POINT('Ctrl Pts',(18.5408278888795,17.1028144183628,-18.1245815961476));
#91398=CARTESIAN_POINT('Ctrl Pts',(18.5323261262762,17.1036107234177,-18.1250887565259));
#91399=CARTESIAN_POINT('Ctrl Pts',(18.5051985080918,17.1063172591723,-18.1267028665239));
#91400=CARTESIAN_POINT('Ctrl Pts',(18.4865927541825,17.108423188016,-18.1278036599205));
#91401=CARTESIAN_POINT('Ctrl Pts',(18.443284526461,17.1139079618984,-18.1303528216572));
#91402=CARTESIAN_POINT('Ctrl Pts',(18.4186086918266,17.1174769170304,-18.1317952476117));
#91403=CARTESIAN_POINT('Ctrl Pts',(18.332072820792,17.1315577262709,-18.1368249801372));
#91404=CARTESIAN_POINT('Ctrl Pts',(18.2706204225959,17.1443829852342,-18.1403437948504));
#91405=CARTESIAN_POINT('Ctrl Pts',(18.0890101236765,17.1907954277338,-18.1507066446127));
#91406=CARTESIAN_POINT('Ctrl Pts',(17.9711630272875,17.2322838473503,-18.1573707516173));
#91407=CARTESIAN_POINT('Ctrl Pts',(17.7746724313688,17.3216378176537,-18.1692247103236));
#91408=CARTESIAN_POINT('Ctrl Pts',(17.694225304787,17.3646892892378,-18.1743222554369));
#91409=CARTESIAN_POINT('Ctrl Pts',(17.6087795695628,17.4177745718916,-18.1802822045596));
#91410=CARTESIAN_POINT('Ctrl Pts',(17.6007795166221,17.4228194214088,-18.1808457704524));
#91411=CARTESIAN_POINT('Ctrl Pts',(17.5889454065238,17.4303933418688,-18.18168812737));
#91412=CARTESIAN_POINT('Ctrl Pts',(17.58508521665,17.4328816370354,-18.1819642842158));
#91413=CARTESIAN_POINT('Ctrl Pts',(17.5782984602636,17.437287736454,-18.1824523120774));
#91414=CARTESIAN_POINT('Ctrl Pts',(17.5753685121989,17.4392002601475,-18.1826638296609));
#91415=CARTESIAN_POINT('Ctrl Pts',(17.5724154762232,17.4411383118368,-18.1828778616448));
#91416=CARTESIAN_POINT('Ctrl Pts',(17.5723876768811,17.4411565572391,-18.1828798765785));
#91417=CARTESIAN_POINT('Ctrl Pts',(17.5723329295829,17.4411924911032,-18.1828838448852));
#91418=CARTESIAN_POINT('Ctrl Pts',(17.5723059815571,17.4412101795543,-18.1828857982588));
#91419=CARTESIAN_POINT('Ctrl Pts',(17.5722528731422,17.4412450411944,-18.1828896480527));
#91420=CARTESIAN_POINT('Ctrl Pts',(17.5722267126976,17.4412622143691,-18.182891544473));
#91421=CARTESIAN_POINT('Ctrl Pts',(17.572175122085,17.441296082961,-18.1828952845066));
#91422=CARTESIAN_POINT('Ctrl Pts',(17.5721496918833,17.4413127783547,-18.1828971281186));
#91423=CARTESIAN_POINT('Ctrl Pts',(17.5720995102198,17.4413457250849,-18.1829007662609));
#91424=CARTESIAN_POINT('Ctrl Pts',(17.5720747586255,17.4413619764671,-18.1829025607975));
#91425=CARTESIAN_POINT('Ctrl Pts',(17.5720258872356,17.4413940658728,-18.1829061041825));
#91426=CARTESIAN_POINT('Ctrl Pts',(17.5720017674302,17.4414099038655,-18.1829078530285));
#91427=CARTESIAN_POINT('Ctrl Pts',(17.5719541167089,17.4414411945576,-18.1829113081347));
#91428=CARTESIAN_POINT('Ctrl Pts',(17.571930585955,17.4414566471167,-18.1829130143804));
#91429=CARTESIAN_POINT('Ctrl Pts',(17.5718840751017,17.4414871919498,-18.18291638705));
#91430=CARTESIAN_POINT('Ctrl Pts',(17.5718610948154,17.4415022843157,-18.1829180534851));
#91431=CARTESIAN_POINT('Ctrl Pts',(17.571815648977,17.4415321322613,-18.1829213491311));
#91432=CARTESIAN_POINT('Ctrl Pts',(17.5717931835544,17.4415468877278,-18.1829229783303));
#91433=CARTESIAN_POINT('Ctrl Pts',(17.5717487348362,17.4415760832076,-18.1829262018624));
#91434=CARTESIAN_POINT('Ctrl Pts',(17.5717267516314,17.4415905231353,-18.1829277961867));
#91435=CARTESIAN_POINT('Ctrl Pts',(17.5716832380417,17.4416191067115,-18.1829309520881));
#91436=CARTESIAN_POINT('Ctrl Pts',(17.5716617073941,17.4416332505086,-18.1829325136824));
#91437=CARTESIAN_POINT('Ctrl Pts',(17.5716190706881,17.4416612602982,-18.1829356061659));
#91438=CARTESIAN_POINT('Ctrl Pts',(17.5715979647949,17.44167512616,-18.1829371370414));
#91439=CARTESIAN_POINT('Ctrl Pts',(17.5715561524305,17.4417025965481,-18.1829401699072));
#91440=CARTESIAN_POINT('Ctrl Pts',(17.57153544589,17.4417162010995,-18.182941671901));
#91441=CARTESIAN_POINT('Ctrl Pts',(17.5714944086082,17.4417431643273,-18.1829446487124));
#91442=CARTESIAN_POINT('Ctrl Pts',(17.5714740778194,17.4417565230162,-18.1829461235319));
#91443=CARTESIAN_POINT('Ctrl Pts',(17.5714337701556,17.4417830088435,-18.1829490475778));
#91444=CARTESIAN_POINT('Ctrl Pts',(17.5714137932678,17.4417961359732,-18.1829504968036));
#91445=CARTESIAN_POINT('Ctrl Pts',(17.5713741726683,17.441822172258,-18.1829533711625));
#91446=CARTESIAN_POINT('Ctrl Pts',(17.5713545291607,17.4418350812631,-18.1829547962794));
#91447=CARTESIAN_POINT('Ctrl Pts',(17.5713155565373,17.4418606935957,-18.1829576237793));
#91448=CARTESIAN_POINT('Ctrl Pts',(17.5712962274227,17.4418733969075,-18.182959026161));
#91449=CARTESIAN_POINT('Ctrl Pts',(17.5712578661399,17.441898609275,-18.1829618094526));
#91450=CARTESIAN_POINT('Ctrl Pts',(17.5712388337983,17.4419111184308,-18.182963190374));
#91451=CARTESIAN_POINT('Ctrl Pts',(17.5712010491702,17.441935953547,-18.1829659319673));
#91452=CARTESIAN_POINT('Ctrl Pts',(17.5711822968948,17.4419482794874,-18.1829672926374));
#91453=CARTESIAN_POINT('Ctrl Pts',(17.5711450571503,17.4419727581579,-18.1829699948314));
#91454=CARTESIAN_POINT('Ctrl Pts',(17.5711265695495,17.4419849109626,-18.1829713363639));
#91455=CARTESIAN_POINT('Ctrl Pts',(17.5710898439478,17.4420090533225,-18.1829740013835));
#91456=CARTESIAN_POINT('Ctrl Pts',(17.5710716061683,17.4420210427209,-18.1829753248536));
#91457=CARTESIAN_POINT('Ctrl Pts',(17.5710353669697,17.4420448669384,-18.1829779547063));
#91458=CARTESIAN_POINT('Ctrl Pts',(17.5710173653863,17.4420567018553,-18.1829792611));
#91459=CARTESIAN_POINT('Ctrl Pts',(17.5709815858628,17.4420802254397,-18.1829818577204));
#91460=CARTESIAN_POINT('Ctrl Pts',(17.5709638077115,17.4420919142364,-18.1829831479616));
#91461=CARTESIAN_POINT('Ctrl Pts',(17.5709284620844,17.4421151540779,-18.1829857132159));
#91462=CARTESIAN_POINT('Ctrl Pts',(17.5709108948849,17.442126704932,-18.1829869882081));
#91463=CARTESIAN_POINT('Ctrl Pts',(17.5708759600353,17.4421496761772,-18.1829895237697));
#91464=CARTESIAN_POINT('Ctrl Pts',(17.5708585923436,17.4421610965871,-18.1829907843414));
#91465=CARTESIAN_POINT('Ctrl Pts',(17.5708240457307,17.4421838140066,-18.1829932918422));
#91466=CARTESIAN_POINT('Ctrl Pts',(17.5708068667396,17.4421951110542,-18.1829945387758));
#91467=CARTESIAN_POINT('Ctrl Pts',(17.5707726865593,17.4422175889388,-18.1829970197947));
#91468=CARTESIAN_POINT('Ctrl Pts',(17.5707556856181,17.4422287696052,-18.1829982538614));
#91469=CARTESIAN_POINT('Ctrl Pts',(17.5707218526017,17.4422510205822,-18.1830007097934));
#91470=CARTESIAN_POINT('Ctrl Pts',(17.5707050202001,17.4422620911005,-18.1830019316819));
#91471=CARTESIAN_POINT('Ctrl Pts',(17.5706715144529,17.4422841282125,-18.1830043639678));
#91472=CARTESIAN_POINT('Ctrl Pts',(17.5706548411569,17.4422950947672,-18.1830055743611));
#91473=CARTESIAN_POINT('Ctrl Pts',(17.5706216444584,17.4423169299593,-18.1830079843205));
#91474=CARTESIAN_POINT('Ctrl Pts',(17.570605121206,17.4423277984921,-18.1830091838751));
#91475=CARTESIAN_POINT('Ctrl Pts',(17.570572216745,17.4423494427856,-18.1830115727255));
#91476=CARTESIAN_POINT('Ctrl Pts',(17.5705558352775,17.4423602187111,-18.1830127620395));
#91477=CARTESIAN_POINT('Ctrl Pts',(17.5705232060589,17.4423816832514,-18.183015131012));
#91478=CARTESIAN_POINT('Ctrl Pts',(17.5705069582918,17.4423923718713,-18.183016310671));
#91479=CARTESIAN_POINT('Ctrl Pts',(17.566982828392,17.4447107960331,-18.1832721835445));
#91480=CARTESIAN_POINT('Ctrl Pts',(17.56348185495,17.4470289395001,-18.183527578501));
#91481=CARTESIAN_POINT('Ctrl Pts',(17.5533919580001,17.45375315368,-18.1842670607959));
#91482=CARTESIAN_POINT('Ctrl Pts',(17.5468209376607,17.4581857779186,-18.1847528846693));
#91483=CARTESIAN_POINT('Ctrl Pts',(17.5033266597986,17.4878825520949,-18.1879960317687));
#91484=CARTESIAN_POINT('Ctrl Pts',(17.467190127829,17.5142729428558,-18.190822405644));
#91485=CARTESIAN_POINT('Ctrl Pts',(17.3385925468834,17.6145862361737,-18.2012934831911));
#91486=CARTESIAN_POINT('Ctrl Pts',(17.251538945909,17.6950823624554,-18.2091816948777));
#91487=CARTESIAN_POINT('Ctrl Pts',(17.0719302031485,17.8915077774818,-18.2267169967406));
#91488=CARTESIAN_POINT('Ctrl Pts',(16.983870581663,18.0107508526359,-18.2362464651292));
#91489=CARTESIAN_POINT('Ctrl Pts',(16.9017321928617,18.1504877523761,-18.2461429233346));
#91490=CARTESIAN_POINT('Ctrl Pts',(16.8946440500213,18.1628295705175,-18.2470073575586));
#91491=CARTESIAN_POINT('Ctrl Pts',(16.8835524970935,18.1826011299718,-18.2483771351266));
#91492=CARTESIAN_POINT('Ctrl Pts',(16.8794682167216,18.1899847871268,-18.2488853765757));
#91493=CARTESIAN_POINT('Ctrl Pts',(16.8723380095826,18.2030588869045,-18.2497795699371));
#91494=CARTESIAN_POINT('Ctrl Pts',(16.8692737762323,18.2087391727414,-18.2501661725114));
#91495=CARTESIAN_POINT('Ctrl Pts',(16.8629851028918,18.2205254005149,-18.2509644709339));
#91496=CARTESIAN_POINT('Ctrl Pts',(16.8597644601158,18.2266332897756,-18.251376028527));
#91497=CARTESIAN_POINT('Ctrl Pts',(16.8515648039321,18.2423699197297,-18.252430966219));
#91498=CARTESIAN_POINT('Ctrl Pts',(16.846629717173,18.2520214173842,-18.2530727921898));
#91499=CARTESIAN_POINT('Ctrl Pts',(16.826264297891,18.2926160735764,-18.2557511773201));
#91500=CARTESIAN_POINT('Ctrl Pts',(16.8115185774839,18.3238980178994,-18.2577638058596));
#91501=CARTESIAN_POINT('Ctrl Pts',(16.7787536063524,18.3980651762211,-18.2624275038487));
#91502=CARTESIAN_POINT('Ctrl Pts',(16.7613690522028,18.4412087662872,-18.2650577862056));
#91503=CARTESIAN_POINT('Ctrl Pts',(16.7454194512262,18.4848895393686,-18.2676549287063));
#91504=CARTESIAN_POINT('Ctrl Pts',(16.7454193875989,18.4848897136231,-18.0457833433865));
#91505=CARTESIAN_POINT('Ctrl Pts',(16.7694007750431,18.4192124700628,-18.0412352318572));
#91506=CARTESIAN_POINT('Ctrl Pts',(16.7966314900153,18.3547353160456,-18.0366093750544));
#91507=CARTESIAN_POINT('Ctrl Pts',(16.8579483854115,18.2275406538387,-18.0272786197108));
#91508=CARTESIAN_POINT('Ctrl Pts',(16.892096831064,18.1649811270577,-18.0225819649794));
#91509=CARTESIAN_POINT('Ctrl Pts',(16.978591243529,18.0239422161366,-18.011832929093));
#91510=CARTESIAN_POINT('Ctrl Pts',(17.0331590482315,17.9469943678683,-18.0058472848897));
#91511=CARTESIAN_POINT('Ctrl Pts',(17.1062782688705,17.8572369002143,-17.9987333372101));
#91512=CARTESIAN_POINT('Ctrl Pts',(17.120130926287,17.8407521278998,-17.9974205295563));
#91513=CARTESIAN_POINT('Ctrl Pts',(17.1388605828479,17.8191418315462,-17.9956905478605));
#91514=CARTESIAN_POINT('Ctrl Pts',(17.1435148395733,17.8138257525991,-17.9952642363448));
#91515=CARTESIAN_POINT('Ctrl Pts',(17.1527788562823,17.8033506982318,-17.9944226994679));
#91516=CARTESIAN_POINT('Ctrl Pts',(17.1573874620078,17.7981908235994,-17.9940074335443));
#91517=CARTESIAN_POINT('Ctrl Pts',(17.1663406818436,17.7882650107935,-17.9932071352293));
#91518=CARTESIAN_POINT('Ctrl Pts',(17.1706819361164,17.7834961576686,-17.992821968023));
#91519=CARTESIAN_POINT('Ctrl Pts',(17.1807318671667,17.7725571736575,-17.9919368744562));
#91520=CARTESIAN_POINT('Ctrl Pts',(17.1864556614052,17.7664010313155,-17.9914375981433));
#91521=CARTESIAN_POINT('Ctrl Pts',(17.2018931563937,17.7499945110545,-17.9901037071673));
#91522=CARTESIAN_POINT('Ctrl Pts',(17.2116731110691,17.7398068527246,-17.9892719465976));
#91523=CARTESIAN_POINT('Ctrl Pts',(17.2964936087109,17.6532019038836,-17.9821687483938));
#91524=CARTESIAN_POINT('Ctrl Pts',(17.3771357592124,17.5824781851315,-17.9761599972751));
#91525=CARTESIAN_POINT('Ctrl Pts',(17.557081758988,17.4473515974383,-17.9637965954818));
#91526=CARTESIAN_POINT('Ctrl Pts',(17.6571165237939,17.3845518013112,-17.9574902290854));
#91527=CARTESIAN_POINT('Ctrl Pts',(17.8135386826446,17.3036917516068,-17.9477841101837));
#91528=CARTESIAN_POINT('Ctrl Pts',(17.8662965452217,17.279119169192,-17.9445320299065));
#91529=CARTESIAN_POINT('Ctrl Pts',(17.9471276805199,17.2454504963471,-17.9394869599092));
#91530=CARTESIAN_POINT('Ctrl Pts',(17.974491093388,17.2347158800626,-17.9377685758654));
#91531=CARTESIAN_POINT('Ctrl Pts',(18.0086259090111,17.2221384461147,-17.9356016719268));
#91532=CARTESIAN_POINT('Ctrl Pts',(18.0151961434791,17.2197544437846,-17.9351835322876));
#91533=CARTESIAN_POINT('Ctrl Pts',(18.025625938475,17.2160283496411,-17.9345179139001));
#91534=CARTESIAN_POINT('Ctrl Pts',(18.02947785329,17.2146647974544,-17.9342716903632));
#91535=CARTESIAN_POINT('Ctrl Pts',(18.0367077138852,17.2121290055456,-17.9338087516652));
#91536=CARTESIAN_POINT('Ctrl Pts',(18.0400846899702,17.2109541688816,-17.9335921930797));
#91537=CARTESIAN_POINT('Ctrl Pts',(18.047829942678,17.208281603055,-17.9330947703364));
#91538=CARTESIAN_POINT('Ctrl Pts',(18.0522001418168,17.2067896124719,-17.9328135718565));
#91539=CARTESIAN_POINT('Ctrl Pts',(18.0657524619673,17.2022122911968,-17.9319399868914));
#91540=CARTESIAN_POINT('Ctrl Pts',(18.0749507521021,17.1991757254206,-17.9313448401075));
#91541=CARTESIAN_POINT('Ctrl Pts',(18.1838239490618,17.164060961566,-17.9242770427483));
#91542=CARTESIAN_POINT('Ctrl Pts',(18.2857145920554,17.1393610118921,-17.9174370809357));
#91543=CARTESIAN_POINT('Ctrl Pts',(18.5556538025838,17.0947739039101,-17.8993941173019));
#91544=CARTESIAN_POINT('Ctrl Pts',(18.725034735708,17.0872867813506,-17.888201308236));
#91545=CARTESIAN_POINT('Ctrl Pts',(18.9210776613035,17.1021010602245,-17.8759055917875));
#91546=CARTESIAN_POINT('Ctrl Pts',(18.9485933595457,17.1047230497041,-17.8741931402574));
#91547=CARTESIAN_POINT('Ctrl Pts',(18.9960376606,17.1101834854926,-17.8712628653616));
#91548=CARTESIAN_POINT('Ctrl Pts',(19.015991160724,17.1127686513795,-17.8700373715249));
#91549=CARTESIAN_POINT('Ctrl Pts',(19.0447123268009,17.1169068732953,-17.8682828198744));
#91550=CARTESIAN_POINT('Ctrl Pts',(19.0535113359188,17.1182313354469,-17.8677465748083));
#91551=CARTESIAN_POINT('Ctrl Pts',(19.0687294139861,17.1206202375685,-17.8668212701996));
#91552=CARTESIAN_POINT('Ctrl Pts',(19.0751523578311,17.1216588593569,-17.8664313983205));
#91553=CARTESIAN_POINT('Ctrl Pts',(19.0874780352979,17.1237103352193,-17.8656844677823));
#91554=CARTESIAN_POINT('Ctrl Pts',(19.0933814501789,17.1247186573857,-17.8653272693811));
#91555=CARTESIAN_POINT('Ctrl Pts',(19.1088023277615,17.1274199892045,-17.864395582684));
#91556=CARTESIAN_POINT('Ctrl Pts',(19.1183126826966,17.1291531725628,-17.8638223758359));
#91557=CARTESIAN_POINT('Ctrl Pts',(19.1511148014039,17.1353635245841,-17.86184984785));
#91558=CARTESIAN_POINT('Ctrl Pts',(19.1743435098283,17.1401670285286,-17.8604609163047));
#91559=CARTESIAN_POINT('Ctrl Pts',(19.3559695113042,17.1809201832999,-17.8496523143701));
#91560=CARTESIAN_POINT('Ctrl Pts',(19.5098343618125,17.2345996954044,-17.84086054137));
#91561=CARTESIAN_POINT('Ctrl Pts',(19.7732432839508,17.3620519303113,-17.8249632570808));
#91562=CARTESIAN_POINT('Ctrl Pts',(19.8849297401308,17.4294314593247,-17.8178826643024));
#91563=CARTESIAN_POINT('Ctrl Pts',(19.9992785490981,17.5136784059995,-17.8095008712134));
#91564=CARTESIAN_POINT('Ctrl Pts',(20.0087921745942,17.5208120526872,-17.8087942035455));
#91565=CARTESIAN_POINT('Ctrl Pts',(20.0222355116379,17.5310703991321,-17.8077815124583));
#91566=CARTESIAN_POINT('Ctrl Pts',(20.0262151820152,17.5341296652678,-17.807479940922));
#91567=CARTESIAN_POINT('Ctrl Pts',(20.0330563060198,17.5394274133314,-17.8069583822628));
#91568=CARTESIAN_POINT('Ctrl Pts',(20.0359229770487,17.5416591838708,-17.8067388697597));
#91569=CARTESIAN_POINT('Ctrl Pts',(20.0414713245671,17.5460016871227,-17.8063121160466));
#91570=CARTESIAN_POINT('Ctrl Pts',(20.0441536477917,17.548111529523,-17.8061049430936));
#91571=CARTESIAN_POINT('Ctrl Pts',(20.0513796124041,17.553823612937,-17.8055445352819));
#91572=CARTESIAN_POINT('Ctrl Pts',(20.0559135357071,17.5574380195127,-17.8051904428509));
#91573=CARTESIAN_POINT('Ctrl Pts',(20.0727024771639,17.5709352044647,-17.8038702478292));
#91574=CARTESIAN_POINT('Ctrl Pts',(20.0848616347388,17.5809356865076,-17.8028961890968));
#91575=CARTESIAN_POINT('Ctrl Pts',(20.1982165645823,17.6763054588638,-17.7936543924056));
#91576=CARTESIAN_POINT('Ctrl Pts',(20.2912971904285,17.7708483397255,-17.7848626578304));
#91577=CARTESIAN_POINT('Ctrl Pts',(20.4751312135868,17.9963798255623,-17.7656435836203));
#91578=CARTESIAN_POINT('Ctrl Pts',(20.5612183200509,18.1301987969987,-17.7553219516416));
#91579=CARTESIAN_POINT('Ctrl Pts',(20.6409909805632,18.291474473976,-17.7442711325658));
#91580=CARTESIAN_POINT('Ctrl Pts',(20.6501374156965,18.3106893597136,-17.7429741982922));
#91581=CARTESIAN_POINT('Ctrl Pts',(20.6627342311604,18.3382147464022,-17.7411435616999));
#91582=CARTESIAN_POINT('Ctrl Pts',(20.6664235295409,18.3464138910887,-17.7406016492379));
#91583=CARTESIAN_POINT('Ctrl Pts',(20.6726991486793,18.360601764511,-17.7396696763341));
#91584=CARTESIAN_POINT('Ctrl Pts',(20.6753102072901,18.3665793533067,-17.7392787715828));
#91585=CARTESIAN_POINT('Ctrl Pts',(20.680257491221,18.3780495795848,-17.7385319856521));
#91586=CARTESIAN_POINT('Ctrl Pts',(20.6825981929262,18.3835402072292,-17.7381759545686));
#91587=CARTESIAN_POINT('Ctrl Pts',(20.6886261004958,18.3978474111791,-17.7372519347542));
#91588=CARTESIAN_POINT('Ctrl Pts',(20.6922769106077,18.4066792484475,-17.7366851858077));
#91589=CARTESIAN_POINT('Ctrl Pts',(20.7045303054971,18.4369000123294,-17.7347580499153));
#91590=CARTESIAN_POINT('Ctrl Pts',(20.7128434507132,18.4584050659376,-17.7334074117917));
#91591=CARTESIAN_POINT('Ctrl Pts',(20.7810962753581,18.6439219186914,-17.7219216025564));
#91592=CARTESIAN_POINT('Ctrl Pts',(20.8208822866533,18.8146292509893,-17.7125287212828));
#91593=CARTESIAN_POINT('Ctrl Pts',(20.8484696836762,19.0754196754077,-17.6982616249294));
#91594=CARTESIAN_POINT('Ctrl Pts',(20.8522681123727,19.1630224933138,-17.6934673595822));
#91595=CARTESIAN_POINT('Ctrl Pts',(20.8499192066847,19.2885696708907,-17.6862991722787));
#91596=CARTESIAN_POINT('Ctrl Pts',(20.8481873581345,19.3265099738846,-17.6840935315199));
#91597=CARTESIAN_POINT('Ctrl Pts',(20.8448871336712,19.3719408934137,-17.681383442228));
#91598=CARTESIAN_POINT('Ctrl Pts',(20.8442973265724,19.3794982249009,-17.6809303278143));
#91599=CARTESIAN_POINT('Ctrl Pts',(20.8433189958267,19.3912217550084,-17.6802236297753));
#91600=CARTESIAN_POINT('Ctrl Pts',(20.8429586795066,19.3953903321004,-17.6799716020201));
#91601=CARTESIAN_POINT('Ctrl Pts',(20.8422686044159,19.4031072385222,-17.6795036217923));
#91602=CARTESIAN_POINT('Ctrl Pts',(20.8419422433812,19.4066558137334,-17.6792878618748));
#91603=CARTESIAN_POINT('Ctrl Pts',(20.8411855869811,19.4146613651401,-17.6787998455118));
#91604=CARTESIAN_POINT('Ctrl Pts',(20.8407501125497,19.4191177840819,-17.6785273028526));
#91605=CARTESIAN_POINT('Ctrl Pts',(20.8394274758862,19.4322232757449,-17.6777232822785));
#91606=CARTESIAN_POINT('Ctrl Pts',(20.8385011777521,19.4408681814495,-17.6771896825332));
#91607=CARTESIAN_POINT('Ctrl Pts',(20.8315687415822,19.5020090784442,-17.6733940694801));
#91608=CARTESIAN_POINT('Ctrl Pts',(20.8236527906456,19.5542653691349,-17.6700368099673));
#91609=CARTESIAN_POINT('Ctrl Pts',(20.8085615198715,19.6336920229547,-17.6648134546291));
#91610=CARTESIAN_POINT('Ctrl Pts',(20.8027856594876,19.6611109320709,-17.6629879272846));
#91611=CARTESIAN_POINT('Ctrl Pts',(20.7654794458532,19.8222794246022,-17.6521522063743));
#91612=CARTESIAN_POINT('Ctrl Pts',(20.721527248678,19.9528296853035,-17.6429724273416));
#91613=CARTESIAN_POINT('Ctrl Pts',(20.6398198646363,20.1347899396232,-17.6300832910823));
#91614=CARTESIAN_POINT('Ctrl Pts',(20.6119317713591,20.1902398138991,-17.6261368762026));
#91615=CARTESIAN_POINT('Ctrl Pts',(20.56341174853,20.2769911100224,-17.6199428209381));
#91616=CARTESIAN_POINT('Ctrl Pts',(20.544316817235,20.3091064121426,-17.6176448544003));
#91617=CARTESIAN_POINT('Ctrl Pts',(20.5184335733051,20.3501268746623,-17.6147012688758));
#91618=CARTESIAN_POINT('Ctrl Pts',(20.5124117314167,20.3595055224583,-17.61402766517));
#91619=CARTESIAN_POINT('Ctrl Pts',(20.5025027569214,20.3746733262951,-17.6129371575771));
#91620=CARTESIAN_POINT('Ctrl Pts',(20.4986606520937,20.380491511868,-17.6125185834845));
#91621=CARTESIAN_POINT('Ctrl Pts',(20.491220098872,20.3916387547516,-17.6117160633738));
#91622=CARTESIAN_POINT('Ctrl Pts',(20.4876259826827,20.3969705980208,-17.6113319605348));
#91623=CARTESIAN_POINT('Ctrl Pts',(20.4793459026301,20.4091340941558,-17.6104550931246));
#91624=CARTESIAN_POINT('Ctrl Pts',(20.4746440004502,20.4159548099744,-17.6099629389182));
#91625=CARTESIAN_POINT('Ctrl Pts',(20.4620569814684,20.4339864768083,-17.6086605316839));
#91626=CARTESIAN_POINT('Ctrl Pts',(20.4541027413163,20.4451488670963,-17.6078529222034));
#91627=CARTESIAN_POINT('Ctrl Pts',(20.3933247531992,20.5287110139857,-17.601794959091));
#91628=CARTESIAN_POINT('Ctrl Pts',(20.3360564619037,20.5977728215801,-17.5967243210894));
#91629=CARTESIAN_POINT('Ctrl Pts',(20.1788940193098,20.7645223122779,-17.5840353610477));
#91630=CARTESIAN_POINT('Ctrl Pts',(20.0734157494003,20.8563309625267,-17.5766145748611));
#91631=CARTESIAN_POINT('Ctrl Pts',(19.9142050327264,20.969384287177,-17.5658324970017));
#91632=CARTESIAN_POINT('Ctrl Pts',(19.8674784146453,20.9998613797976,-17.5627088847467));
#91633=CARTESIAN_POINT('Ctrl Pts',(19.7950134452223,21.0431463104387,-17.5578409965815));
#91634=CARTESIAN_POINT('Ctrl Pts',(19.7701258074578,21.0573349539123,-17.5561650477678));
#91635=CARTESIAN_POINT('Ctrl Pts',(19.7388474017694,21.0743354746634,-17.5540440287497));
#91636=CARTESIAN_POINT('Ctrl Pts',(19.7327191813931,21.0776272754986,-17.5536277773761));
#91637=CARTESIAN_POINT('Ctrl Pts',(19.7230001955002,21.0827863106764,-17.5529663610738));
#91638=CARTESIAN_POINT('Ctrl Pts',(19.7194200456824,21.0846735874935,-17.5527224470012));
#91639=CARTESIAN_POINT('Ctrl Pts',(19.7126603391451,21.0882122355443,-17.5522613605475));
#91640=CARTESIAN_POINT('Ctrl Pts',(19.7094819942835,21.0898658054284,-17.5520443299069));
#91641=CARTESIAN_POINT('Ctrl Pts',(19.7022091732893,21.0936261445186,-17.5515471936676));
#91642=CARTESIAN_POINT('Ctrl Pts',(19.6981120162057,21.0957276255603,-17.5512667602578));
#91643=CARTESIAN_POINT('Ctrl Pts',(19.6872234748587,21.101267693771,-17.5505205684744));
#91644=CARTESIAN_POINT('Ctrl Pts',(19.6804204159355,21.104683009228,-17.5500534125796));
#91645=CARTESIAN_POINT('Ctrl Pts',(19.6328499252083,21.1282442881864,-17.5467810402348));
#91646=CARTESIAN_POINT('Ctrl Pts',(19.5914641285686,21.1471072908906,-17.5439048049551));
#91647=CARTESIAN_POINT('Ctrl Pts',(19.5442245208114,21.1668266768969,-17.5406145969368));
#91648=CARTESIAN_POINT('Ctrl Pts',(19.5389333864481,21.1690102161501,-17.540245970546));
#91649=CARTESIAN_POINT('Ctrl Pts',(19.3878102258,21.2306594626412,-17.5297157049605));
#91650=CARTESIAN_POINT('Ctrl Pts',(19.2358040147326,21.2736896493362,-17.5191256584674));
#91651=CARTESIAN_POINT('Ctrl Pts',(18.9788178326079,21.3163173978165,-17.5022143764419));
#91652=CARTESIAN_POINT('Ctrl Pts',(18.8761048670814,21.3257361038233,-17.4956952021538));
#91653=CARTESIAN_POINT('Ctrl Pts',(18.7582952652666,21.327912374419,-17.4885096331805));
#91654=CARTESIAN_POINT('Ctrl Pts',(18.7434875837209,21.3280305298032,-17.4876115088568));
#91655=CARTESIAN_POINT('Ctrl Pts',(18.7209109523997,21.3279737902928,-17.4862496142555));
#91656=CARTESIAN_POINT('Ctrl Pts',(18.7131424119755,21.3279115039332,-17.4857823326196));
#91657=CARTESIAN_POINT('Ctrl Pts',(18.6990135014297,21.3277204378913,-17.4849348580076));
#91658=CARTESIAN_POINT('Ctrl Pts',(18.6926530611768,21.327605749611,-17.4845542283781));
#91659=CARTESIAN_POINT('Ctrl Pts',(18.6789274053218,21.3272963619309,-17.4837346994523));
#91660=CARTESIAN_POINT('Ctrl Pts',(18.6715624771499,21.3270918789247,-17.4832961114984));
#91661=CARTESIAN_POINT('Ctrl Pts',(18.6516067753745,21.3264335455224,-17.4821107794829));
#91662=CARTESIAN_POINT('Ctrl Pts',(18.6390186167652,21.3259057369416,-17.4813663563354));
#91663=CARTESIAN_POINT('Ctrl Pts',(18.5779499495872,21.3227988388268,-17.4777700569275));
#91664=CARTESIAN_POINT('Ctrl Pts',(18.5295609840548,21.3186648628839,-17.4749671559836));
#91665=CARTESIAN_POINT('Ctrl Pts',(18.4408402631761,21.3080005841054,-17.4698882905772));
#91666=CARTESIAN_POINT('Ctrl Pts',(18.4004744140076,21.3019603081542,-17.46760061205));
#91667=CARTESIAN_POINT('Ctrl Pts',(18.2279671705293,21.2710235012372,-17.4578738607842));
#91668=CARTESIAN_POINT('Ctrl Pts',(18.0981936382654,21.234738032034,-17.4507040386991));
#91669=CARTESIAN_POINT('Ctrl Pts',(17.914208005236,21.1638350443407,-17.4398677489502));
#91670=CARTESIAN_POINT('Ctrl Pts',(17.8567128101947,21.1386902401825,-17.4363742131181));
#91671=CARTESIAN_POINT('Ctrl Pts',(17.7726606707444,21.0973914040426,-17.4309874992658));
#91672=CARTESIAN_POINT('Ctrl Pts',(17.7452021041984,21.0831443131641,-17.4291811176432));
#91673=CARTESIAN_POINT('Ctrl Pts',(17.711812846052,21.0648805902241,-17.4269145474043));
#91674=CARTESIAN_POINT('Ctrl Pts',(17.7055759333888,21.0614279927707,-17.4264881055031));
#91675=CARTESIAN_POINT('Ctrl Pts',(17.6957925211661,21.0559474032014,-17.4258141591422));
#91676=CARTESIAN_POINT('Ctrl Pts',(17.6922341846518,21.0539404968716,-17.4255679869908));
#91677=CARTESIAN_POINT('Ctrl Pts',(17.6855723010471,21.0501577272888,-17.4251050905651));
#91678=CARTESIAN_POINT('Ctrl Pts',(17.682467436557,21.0483842965251,-17.4248885225401));
#91679=CARTESIAN_POINT('Ctrl Pts',(17.6753618172859,21.0443018125396,-17.424391005736));
#91680=CARTESIAN_POINT('Ctrl Pts',(17.6713641286261,21.0419875318245,-17.4241097221638));
#91681=CARTESIAN_POINT('Ctrl Pts',(17.6590006518283,21.0347761293966,-17.423235615169));
#91682=CARTESIAN_POINT('Ctrl Pts',(17.650661039943,21.0298346978623,-17.4226400267852));
#91683=CARTESIAN_POINT('Ctrl Pts',(17.560183280674,20.9753813171494,-17.4161155796273));
#91684=CARTESIAN_POINT('Ctrl Pts',(17.4814756293523,20.9204050057408,-17.4098775552118));
#91685=CARTESIAN_POINT('Ctrl Pts',(17.3080590803382,20.7808525208292,-17.3952245813983));
#91686=CARTESIAN_POINT('Ctrl Pts',(17.2166658943002,20.6927037832022,-17.3867948010584));
#91687=CARTESIAN_POINT('Ctrl Pts',(17.0955502260439,20.5528523659937,-17.3748732452443));
#91688=CARTESIAN_POINT('Ctrl Pts',(17.0592305770765,20.5072383169643,-17.371174862511));
#91689=CARTESIAN_POINT('Ctrl Pts',(17.0037578839691,20.4313390331937,-17.3653244384609));
#91690=CARTESIAN_POINT('Ctrl Pts',(16.983411210312,20.4019677869511,-17.3631287167273));
#91691=CARTESIAN_POINT('Ctrl Pts',(16.9578008007423,20.3629226155869,-17.3602956491267));
#91692=CARTESIAN_POINT('Ctrl Pts',(16.9518562841104,20.3537042884106,-17.3596328533288));
#91693=CARTESIAN_POINT('Ctrl Pts',(16.9422715539011,20.3385842517995,-17.3585554693151));
#91694=CARTESIAN_POINT('Ctrl Pts',(16.9385882718256,20.3327102110524,-17.3581392853156));
#91695=CARTESIAN_POINT('Ctrl Pts',(16.9315377850271,20.3213425054804,-17.3573383893286));
#91696=CARTESIAN_POINT('Ctrl Pts',(16.9281666786304,20.315851362279,-17.3569535363394));
#91697=CARTESIAN_POINT('Ctrl Pts',(16.9204737488977,20.3031911953769,-17.356070815532));
#91698=CARTESIAN_POINT('Ctrl Pts',(16.9161692532598,20.2960117280348,-17.3555735863286));
#91699=CARTESIAN_POINT('Ctrl Pts',(16.9047788758154,20.2767556594777,-17.3542487703178));
#91700=CARTESIAN_POINT('Ctrl Pts',(16.8977699551827,20.264633846942,-17.3534239761013));
#91701=CARTESIAN_POINT('Ctrl Pts',(16.8410121010338,20.164185311981,-17.3466623641973));
#91702=CARTESIAN_POINT('Ctrl Pts',(16.7975427766105,20.0724538047347,-17.3409591108816));
#91703=CARTESIAN_POINT('Ctrl Pts',(16.7062965716862,19.8376978734538,-17.3270884795012));
#91704=CARTESIAN_POINT('Ctrl Pts',(16.6668952196633,19.6920445464143,-17.319119822132));
#91705=CARTESIAN_POINT('Ctrl Pts',(16.6370543890959,19.5043826523554,-17.3084710835149));
#91706=CARTESIAN_POINT('Ctrl Pts',(16.631938189477,19.4651457325877,-17.3062221137651));
#91707=CARTESIAN_POINT('Ctrl Pts',(16.626393979092,19.4107834529683,-17.3030474656015));
#91708=CARTESIAN_POINT('Ctrl Pts',(16.6250239190745,19.3957604686448,-17.3021639816366));
#91709=CARTESIAN_POINT('Ctrl Pts',(16.6229323250509,19.3697556824083,-17.3006220422313));
#91710=CARTESIAN_POINT('Ctrl Pts',(16.6221356451447,19.3587803435252,-17.2999673827355));
#91711=CARTESIAN_POINT('Ctrl Pts',(16.6211102618364,19.3429455002856,-17.2990166282724));
#91712=CARTESIAN_POINT('Ctrl Pts',(16.6208126721346,19.3380904282536,-17.2987242760423));
#91713=CARTESIAN_POINT('Ctrl Pts',(16.6203235173845,19.3296328029661,-17.2982134561621));
#91714=CARTESIAN_POINT('Ctrl Pts',(16.6201244222716,19.3260306778541,-17.2979954101872));
#91715=CARTESIAN_POINT('Ctrl Pts',(16.6197264097696,19.3184793973308,-17.2975372671188));
#91716=CARTESIAN_POINT('Ctrl Pts',(16.6195293495772,19.3145302038257,-17.2972970719183));
#91717=CARTESIAN_POINT('Ctrl Pts',(16.6190357980324,19.3040493179722,-17.2966580762555));
#91718=CARTESIAN_POINT('Ctrl Pts',(16.6187585037377,19.2975168254328,-17.2962582243825));
#91719=CARTESIAN_POINT('Ctrl Pts',(16.6177066689143,19.2696966953738,-17.2945489348637));
#91720=CARTESIAN_POINT('Ctrl Pts',(16.6172232249825,19.2484001290508,-17.2932244436307));
#91721=CARTESIAN_POINT('Ctrl Pts',(16.6170218768569,19.2219269139405,-17.2915610829938));
#91722=CARTESIAN_POINT('Ctrl Pts',(16.6170014935719,19.216752887994,-17.2912351857526));
#91723=CARTESIAN_POINT('Ctrl Pts',(16.6169868170217,19.1630721342973,-17.2878459976942));
#91724=CARTESIAN_POINT('Ctrl Pts',(16.618640710772,19.1145823861424,-17.2847171541311));
#91725=CARTESIAN_POINT('Ctrl Pts',(16.6353861374769,18.8703421461503,-17.2687464404757));
#91726=CARTESIAN_POINT('Ctrl Pts',(16.6759975325268,18.6772599417279,-17.2555537971222));
#91727=CARTESIAN_POINT('Ctrl Pts',(16.7435636729826,18.4899871113246,-17.2430395181198));
#91728=CARTESIAN_POINT('Ctrl Pts',(16.7444891184151,18.4874374185689,-17.2428691684334));
#91729=CARTESIAN_POINT('Ctrl Pts',(16.7454194502294,18.4848895420984,-17.2426989706651));
#91730=CARTESIAN_POINT('Origin',(18.734,19.211,0.));
#91731=CARTESIAN_POINT('',(16.7454194446555,18.4848895573634,-16.4437313838642));
#91732=CARTESIAN_POINT('',(16.7454194503294,18.4848895418246,-16.6645989754405));
#91733=CARTESIAN_POINT('',(16.7454194503191,18.4848895418526,0.));
#91734=CARTESIAN_POINT('',(16.6170007987606,19.2099039755699,-16.7126929344973));
#91735=CARTESIAN_POINT('Ctrl Pts',(16.7454194503294,18.4848895418246,-16.6645989754405));
#91736=CARTESIAN_POINT('Ctrl Pts',(16.7447285761329,18.4867816217058,-16.6647267315824));
#91737=CARTESIAN_POINT('Ctrl Pts',(16.7440404001695,18.4886746935246,-16.664854598572));
#91738=CARTESIAN_POINT('Ctrl Pts',(16.6879393884391,18.6436890726986,-16.6753284307576));
#91739=CARTESIAN_POINT('Ctrl Pts',(16.650376635932,18.8026872523377,-16.6862947866301));
#91740=CARTESIAN_POINT('Ctrl Pts',(16.621854709062,19.0458921890449,-16.7022898980983));
#91741=CARTESIAN_POINT('Ctrl Pts',(16.6170428510048,19.1278576474473,-16.7075611564714));
#91742=CARTESIAN_POINT('Ctrl Pts',(16.617000284921,19.2099016579427,-16.7126936831171));
#91743=CARTESIAN_POINT('Ctrl Pts',(16.6170002837488,19.2099039196303,-16.7126938246042));
#91744=CARTESIAN_POINT('Ctrl Pts',(16.6169868619687,19.2358271140463,-16.7143155325004));
#91745=CARTESIAN_POINT('Ctrl Pts',(16.6174495936211,19.2617494353718,-16.7159232237688));
#91746=CARTESIAN_POINT('Ctrl Pts',(16.6190263313245,19.3052644054436,-16.7185989970965));
#91747=CARTESIAN_POINT('Ctrl Pts',(16.6198840704897,19.3228626987045,-16.7196748128033));
#91748=CARTESIAN_POINT('Ctrl Pts',(16.6214584272066,19.3485615081172,-16.7212369082377));
#91749=CARTESIAN_POINT('Ctrl Pts',(16.6220021593856,19.3566715120544,-16.7217285743142));
#91750=CARTESIAN_POINT('Ctrl Pts',(16.6230473344705,19.3710219815548,-16.722596318813));
#91751=CARTESIAN_POINT('Ctrl Pts',(16.6235297736961,19.3772636938281,-16.7229729894496));
#91752=CARTESIAN_POINT('Ctrl Pts',(16.6245388660994,19.3896063308187,-16.7237163741477));
#91753=CARTESIAN_POINT('Ctrl Pts',(16.6250643169823,19.3957072899552,-16.7240831222323));
#91754=CARTESIAN_POINT('Ctrl Pts',(16.6261638663541,19.4078571848804,-16.7248121146517));
#91755=CARTESIAN_POINT('Ctrl Pts',(16.6267375498195,19.4139060984439,-16.7251743683558));
#91756=CARTESIAN_POINT('Ctrl Pts',(16.6281714408722,19.4283626123967,-16.7260385446406));
#91757=CARTESIAN_POINT('Ctrl Pts',(16.6290559728491,19.4367677377642,-16.7265396984872));
#91758=CARTESIAN_POINT('Ctrl Pts',(16.6319011461661,19.4623317995503,-16.7280601928522));
#91759=CARTESIAN_POINT('Ctrl Pts',(16.6340214751808,19.4794725053514,-16.7290745195657));
#91760=CARTESIAN_POINT('Ctrl Pts',(16.6419661856781,19.5378270006969,-16.7325118270954));
#91761=CARTESIAN_POINT('Ctrl Pts',(16.6487962625818,19.5788954588415,-16.734903562638));
#91762=CARTESIAN_POINT('Ctrl Pts',(16.6900265287536,19.7884237302569,-16.7470133525422));
#91763=CARTESIAN_POINT('Ctrl Pts',(16.7436413625375,19.9524297308197,-16.7561209159006));
#91764=CARTESIAN_POINT('Ctrl Pts',(16.8430671529535,20.1649353143168,-16.769015070992));
#91765=CARTESIAN_POINT('Ctrl Pts',(16.8721436922977,20.2205095627063,-16.772506914072));
#91766=CARTESIAN_POINT('Ctrl Pts',(16.9191779867286,20.3014431519003,-16.7778912675595));
#91767=CARTESIAN_POINT('Ctrl Pts',(16.9352983589405,20.3278336433306,-16.7796970709735));
#91768=CARTESIAN_POINT('Ctrl Pts',(16.955838015451,20.3598602033141,-16.781962996951));
#91769=CARTESIAN_POINT('Ctrl Pts',(16.9597163391459,20.3658408104971,-16.7823893955291));
#91770=CARTESIAN_POINT('Ctrl Pts',(16.9658647090614,20.3752178839487,-16.7830632886657));
#91771=CARTESIAN_POINT('Ctrl Pts',(16.9681145507912,20.3786276238563,-16.7833094512671));
#91772=CARTESIAN_POINT('Ctrl Pts',(16.9723521715327,20.3850096739091,-16.7837723398921));
#91773=CARTESIAN_POINT('Ctrl Pts',(16.9743376166432,20.387983467129,-16.7839889097274));
#91774=CARTESIAN_POINT('Ctrl Pts',(16.978905371257,20.3947876432489,-16.7844864442225));
#91775=CARTESIAN_POINT('Ctrl Pts',(16.9814926832449,20.3986146024436,-16.7847677437638));
#91776=CARTESIAN_POINT('Ctrl Pts',(16.9895487942547,20.4104469497606,-16.7856419485841));
#91777=CARTESIAN_POINT('Ctrl Pts',(16.9950599854416,20.4184231288489,-16.7862376196978));
#91778=CARTESIAN_POINT('Ctrl Pts',(17.0573284912404,20.507231829616,-16.7929389979651));
#91779=CARTESIAN_POINT('Ctrl Pts',(17.1196150372987,20.5840261716636,-16.799372258923));
#91780=CARTESIAN_POINT('Ctrl Pts',(17.3015406323331,20.7787657961343,-16.8169267070101));
#91781=CARTESIAN_POINT('Ctrl Pts',(17.4302425856269,20.8873241182522,-16.8280724108276));
#91782=CARTESIAN_POINT('Ctrl Pts',(17.5967906256836,20.9969003267764,-16.8405985654122));
#91783=CARTESIAN_POINT('Ctrl Pts',(17.6235430601663,21.0136565641113,-16.8425611858813));
#91784=CARTESIAN_POINT('Ctrl Pts',(17.6638282719996,21.0376516766322,-16.8454447101559));
#91785=CARTESIAN_POINT('Ctrl Pts',(17.6770802466514,21.04535125576,-16.8463820183829));
#91786=CARTESIAN_POINT('Ctrl Pts',(17.7013526714543,21.0591034961797,-16.8480787183859));
#91787=CARTESIAN_POINT('Ctrl Pts',(17.7123455617898,21.0652031327013,-16.8488397721356));
#91788=CARTESIAN_POINT('Ctrl Pts',(17.7297375496511,21.0746518119148,-16.8500324566828));
#91789=CARTESIAN_POINT('Ctrl Pts',(17.7361004331576,21.0780665766759,-16.8504664276954));
#91790=CARTESIAN_POINT('Ctrl Pts',(17.7425268566749,21.0814732045099,-16.8509023717785));
#91791=CARTESIAN_POINT('Ctrl Pts',(17.742572988694,21.0814976567688,-16.8509055010767));
#91792=CARTESIAN_POINT('Ctrl Pts',(17.7426668788075,21.0815474187379,-16.850911869727));
#91793=CARTESIAN_POINT('Ctrl Pts',(17.7427146380403,21.0815727288948,-16.8509151091475));
#91794=CARTESIAN_POINT('Ctrl Pts',(17.7428118417404,21.0816242375357,-16.8509217020285));
#91795=CARTESIAN_POINT('Ctrl Pts',(17.7428612873874,21.0816504364768,-16.8509250555596));
#91796=CARTESIAN_POINT('Ctrl Pts',(17.7429619255951,21.0817037548567,-16.8509318808163));
#91797=CARTESIAN_POINT('Ctrl Pts',(17.7430131189639,21.0817308745433,-16.8509353525868));
#91798=CARTESIAN_POINT('Ctrl Pts',(17.743117316422,21.0817860676683,-16.850942418619));
#91799=CARTESIAN_POINT('Ctrl Pts',(17.7431703213666,21.0818141413663,-16.850946012928));
#91800=CARTESIAN_POINT('Ctrl Pts',(17.7432782080578,21.081871276926,-16.8509533284854));
#91801=CARTESIAN_POINT('Ctrl Pts',(17.7433330906024,21.0819003390028,-16.8509570497764));
#91802=CARTESIAN_POINT('Ctrl Pts',(17.7434448009888,21.0819594869601,-16.8509646239069));
#91803=CARTESIAN_POINT('Ctrl Pts',(17.743501629632,21.0819895730421,-16.8509684767885));
#91804=CARTESIAN_POINT('Ctrl Pts',(17.7436173033879,21.0820508060135,-16.8509763188877));
#91805=CARTESIAN_POINT('Ctrl Pts',(17.7436761490008,21.0820819529285,-16.850980308126));
#91806=CARTESIAN_POINT('Ctrl Pts',(17.743795930242,21.0821453457674,-16.8509884278842));
#91807=CARTESIAN_POINT('Ctrl Pts',(17.7438568665135,21.0821775917753,-16.8509925584333));
#91808=CARTESIAN_POINT('Ctrl Pts',(17.7439809051875,21.0822432222997,-16.8510009659292));
#91809=CARTESIAN_POINT('Ctrl Pts',(17.7440440082634,21.0822766068973,-16.8510052429061));
#91810=CARTESIAN_POINT('Ctrl Pts',(17.7441724595007,21.0823445555359,-16.8510139485624));
#91811=CARTESIAN_POINT('Ctrl Pts',(17.7442378082344,21.0823791195843,-16.8510183772639));
#91812=CARTESIAN_POINT('Ctrl Pts',(17.7443708346786,21.0824494705992,-16.8510273920047));
#91813=CARTESIAN_POINT('Ctrl Pts',(17.7444385097022,21.0824852558274,-16.851031977844));
#91814=CARTESIAN_POINT('Ctrl Pts',(17.7445651187777,21.082552195442,-16.8510405567208));
#91815=CARTESIAN_POINT('Ctrl Pts',(17.7446240535157,21.0825833513263,-16.8510445498681));
#91816=CARTESIAN_POINT('Ctrl Pts',(17.7447516740642,21.0826508102924,-16.8510531964201));
#91817=CARTESIAN_POINT('Ctrl Pts',(17.7448203614933,21.0826871129543,-16.8510578498634));
#91818=CARTESIAN_POINT('Ctrl Pts',(17.7449690837388,21.0827657051226,-16.8510679249293));
#91819=CARTESIAN_POINT('Ctrl Pts',(17.745049120253,21.0828079937968,-16.8510733465706));
#91820=CARTESIAN_POINT('Ctrl Pts',(17.7452223905787,21.0828995299494,-16.8510850830394));
#91821=CARTESIAN_POINT('Ctrl Pts',(17.7453156261222,21.082948776,-16.8510913978537));
#91822=CARTESIAN_POINT('Ctrl Pts',(17.7455174346605,21.0830553499014,-16.8511050652072));
#91823=CARTESIAN_POINT('Ctrl Pts',(17.7456260093849,21.0831126754954,-16.8511124176867));
#91824=CARTESIAN_POINT('Ctrl Pts',(17.7458609668928,21.0832367028962,-16.8511283271168));
#91825=CARTESIAN_POINT('Ctrl Pts',(17.7459873511926,21.0833034012196,-16.851136883931));
#91826=CARTESIAN_POINT('Ctrl Pts',(17.7462732744956,21.0834542579886,-16.8511562402255));
#91827=CARTESIAN_POINT('Ctrl Pts',(17.7464328175309,21.0835384088572,-16.8511670394376));
#91828=CARTESIAN_POINT('Ctrl Pts',(17.7523042755597,21.0866343464138,-16.851564415543));
#91829=CARTESIAN_POINT('Ctrl Pts',(17.7580299779621,21.089620029261,-16.8519500648428));
#91830=CARTESIAN_POINT('Ctrl Pts',(17.7712868246782,21.0964558816396,-16.8528387220066));
#91831=CARTESIAN_POINT('Ctrl Pts',(17.7788275936084,21.1002872245328,-16.8533410626657));
#91832=CARTESIAN_POINT('Ctrl Pts',(17.7991801790671,21.1104750438881,-16.8546885773145));
#91833=CARTESIAN_POINT('Ctrl Pts',(17.8120339211277,21.1167471249668,-16.855530803637));
#91834=CARTESIAN_POINT('Ctrl Pts',(17.9304938537348,21.17307150822,-16.8632149735147));
#91835=CARTESIAN_POINT('Ctrl Pts',(18.0400176401703,21.2144321750125,-16.869740077917));
#91836=CARTESIAN_POINT('Ctrl Pts',(18.3090793521164,21.2913078700916,-16.8850589020573));
#91837=CARTESIAN_POINT('Ctrl Pts',(18.4703742342261,21.3178288746519,-16.893668925298));
#91838=CARTESIAN_POINT('Ctrl Pts',(18.6653332390215,21.3271322556068,-16.9048787602948));
#91839=CARTESIAN_POINT('Ctrl Pts',(18.6976032181876,21.3279331273018,-16.9067616839022));
#91840=CARTESIAN_POINT('Ctrl Pts',(18.7371006182579,21.3280100541111,-16.9091134837565));
#91841=CARTESIAN_POINT('Ctrl Pts',(18.744324293872,21.3279871488925,-16.9095455352233));
#91842=CARTESIAN_POINT('Ctrl Pts',(18.7556536680013,21.3278932376672,-16.9102263756007));
#91843=CARTESIAN_POINT('Ctrl Pts',(18.7597595962524,21.3278472556048,-16.9104737864354));
#91844=CARTESIAN_POINT('Ctrl Pts',(18.7674374186014,21.3277389308635,-16.9109377144555));
#91845=CARTESIAN_POINT('Ctrl Pts',(18.7710092974935,21.3276794924209,-16.9111540675673));
#91846=CARTESIAN_POINT('Ctrl Pts',(18.7791669391463,21.3275230889816,-16.9116493745664));
#91847=CARTESIAN_POINT('Ctrl Pts',(18.7837525324062,21.3274202614765,-16.9119286521317));
#91848=CARTESIAN_POINT('Ctrl Pts',(18.7978617023467,21.3270579976204,-16.9127905002145));
#91849=CARTESIAN_POINT('Ctrl Pts',(18.8073837372242,21.3267491783374,-16.9133757272426));
#91850=CARTESIAN_POINT('Ctrl Pts',(18.9364229332486,21.3216920366697,-16.9213521058086));
#91851=CARTESIAN_POINT('Ctrl Pts',(19.0553172939337,21.3068875165682,-16.9292201784027));
#91852=CARTESIAN_POINT('Ctrl Pts',(19.278917930622,21.2595672372516,-16.944319034537));
#91853=CARTESIAN_POINT('Ctrl Pts',(19.3836331873354,21.2288065999973,-16.9515219245795));
#91854=CARTESIAN_POINT('Ctrl Pts',(19.5556696800508,21.1634800837495,-16.9633456297866));
#91855=CARTESIAN_POINT('Ctrl Pts',(19.624359334101,21.1331295334193,-16.9680666263175));
#91856=CARTESIAN_POINT('Ctrl Pts',(19.708074147434,21.0906867550345,-16.9738164859375));
#91857=CARTESIAN_POINT('Ctrl Pts',(19.7247356953516,21.0819584601334,-16.9749608455561));
#91858=CARTESIAN_POINT('Ctrl Pts',(19.7488031797864,21.0689388268045,-16.9766142756146));
#91859=CARTESIAN_POINT('Ctrl Pts',(19.7563025588582,21.0648229849044,-16.9771295418241));
#91860=CARTESIAN_POINT('Ctrl Pts',(19.7694116718697,21.0575246443458,-16.9780304146364));
#91861=CARTESIAN_POINT('Ctrl Pts',(19.7750321554186,21.0543617781739,-16.9784167171584));
#91862=CARTESIAN_POINT('Ctrl Pts',(19.7859209692477,21.0481685309219,-16.9791652647264));
#91863=CARTESIAN_POINT('Ctrl Pts',(19.7911908701844,21.0451410528464,-16.9795276092995));
#91864=CARTESIAN_POINT('Ctrl Pts',(19.8037628120906,21.0378464773464,-16.9803922250094));
#91865=CARTESIAN_POINT('Ctrl Pts',(19.8110524998835,21.0335582134938,-16.9808937256131));
#91866=CARTESIAN_POINT('Ctrl Pts',(19.837294313774,21.0179086609543,-16.9826998326179));
#91867=CARTESIAN_POINT('Ctrl Pts',(19.8560943942174,21.0062942590332,-16.9839952146785));
#91868=CARTESIAN_POINT('Ctrl Pts',(20.0311361676866,20.8943321224197,-16.9960802195306));
#91869=CARTESIAN_POINT('Ctrl Pts',(20.1737155331028,20.7741360980852,-17.0060121270811));
#91870=CARTESIAN_POINT('Ctrl Pts',(20.3527273144784,20.5776831764974,-17.0205012281641));
#91871=CARTESIAN_POINT('Ctrl Pts',(20.4032549682087,20.5154872064165,-17.024905025784));
#91872=CARTESIAN_POINT('Ctrl Pts',(20.4712211668354,20.4213918739281,-17.0315447344727));
#91873=CARTESIAN_POINT('Ctrl Pts',(20.4915579013346,20.3916675003225,-17.0336394527146));
#91874=CARTESIAN_POINT('Ctrl Pts',(20.5151821105899,20.3551743824452,-17.0362265466963));
#91875=CARTESIAN_POINT('Ctrl Pts',(20.5192056544858,20.3488864161047,-17.0366728563519));
#91876=CARTESIAN_POINT('Ctrl Pts',(20.5254189006928,20.3390623299429,-17.037371205983));
#91877=CARTESIAN_POINT('Ctrl Pts',(20.5276316270342,20.3355407435103,-17.0376217485581));
#91878=CARTESIAN_POINT('Ctrl Pts',(20.5317222036078,20.3289877434587,-17.0380883923686));
#91879=CARTESIAN_POINT('Ctrl Pts',(20.533602777282,20.325958097536,-17.0383043101056));
#91880=CARTESIAN_POINT('Ctrl Pts',(20.5378449576885,20.3190851576459,-17.0387945218359));
#91881=CARTESIAN_POINT('Ctrl Pts',(20.5402019285213,20.3152390776044,-17.0390691134711));
#91882=CARTESIAN_POINT('Ctrl Pts',(20.546256291654,20.305288385517,-17.0397801815962));
#91883=CARTESIAN_POINT('Ctrl Pts',(20.5499351028077,20.2991726133277,-17.0402178254077));
#91884=CARTESIAN_POINT('Ctrl Pts',(20.5723467300015,20.2614846619987,-17.0429179787807));
#91885=CARTESIAN_POINT('Ctrl Pts',(20.5902853875496,20.2294502491368,-17.0452267902693));
#91886=CARTESIAN_POINT('Ctrl Pts',(20.6867169475803,20.0462262154028,-17.0584408035116));
#91887=CARTESIAN_POINT('Ctrl Pts',(20.7475691642428,19.8864617645616,-17.0699344876168));
#91888=CARTESIAN_POINT('Ctrl Pts',(20.8116284924949,19.6284529161769,-17.0872115337993));
#91889=CARTESIAN_POINT('Ctrl Pts',(20.8283440005247,19.5343180509846,-17.093278696753));
#91890=CARTESIAN_POINT('Ctrl Pts',(20.8409558166998,19.4180852872211,-17.1004603553849));
#91891=CARTESIAN_POINT('Ctrl Pts',(20.8429419159826,19.3967718426598,-17.1017650198563));
#91892=CARTESIAN_POINT('Ctrl Pts',(20.8453044674437,19.3664466464373,-17.1036045693131));
#91893=CARTESIAN_POINT('Ctrl Pts',(20.8459470682652,19.3574574986415,-17.1041477736253));
#91894=CARTESIAN_POINT('Ctrl Pts',(20.8469560605195,19.3419514584894,-17.1050812699915));
#91895=CARTESIAN_POINT('Ctrl Pts',(20.8473497464858,19.3354365246846,-17.1054724136768));
#91896=CARTESIAN_POINT('Ctrl Pts',(20.8480455185504,19.3229648070265,-17.1062191818024));
#91897=CARTESIAN_POINT('Ctrl Pts',(20.8483525719362,19.3170083731765,-17.1065749584272));
#91898=CARTESIAN_POINT('Ctrl Pts',(20.849084946768,19.3015291665882,-17.1074972936121));
#91899=CARTESIAN_POINT('Ctrl Pts',(20.8494711342402,19.2920046095096,-17.1080626214963));
#91900=CARTESIAN_POINT('Ctrl Pts',(20.8505663755161,19.2595846314874,-17.1099796755452));
#91901=CARTESIAN_POINT('Ctrl Pts',(20.8509681832544,19.2366799480955,-17.1113217929126));
#91902=CARTESIAN_POINT('Ctrl Pts',(20.8512294839296,19.0371639492722,-17.1229163549525));
#91903=CARTESIAN_POINT('Ctrl Pts',(20.8293620856766,18.8612228780746,-17.1324065973639));
#91904=CARTESIAN_POINT('Ctrl Pts',(20.7646788927514,18.6064626451888,-17.1467107748272));
#91905=CARTESIAN_POINT('Ctrl Pts',(20.7383786067801,18.5242786371518,-17.1514330993186));
#91906=CARTESIAN_POINT('Ctrl Pts',(20.6935122575157,18.4088677197828,-17.1585042895766));
#91907=CARTESIAN_POINT('Ctrl Pts',(20.678948685082,18.374173434108,-17.1606900291397));
#91908=CARTESIAN_POINT('Ctrl Pts',(20.6603586941051,18.3329975291665,-17.163378060292));
#91909=CARTESIAN_POINT('Ctrl Pts',(20.6572109417736,18.326123835399,-17.1638299847379));
#91910=CARTESIAN_POINT('Ctrl Pts',(20.6522658673023,18.3154763917768,-17.1645352232892));
#91911=CARTESIAN_POINT('Ctrl Pts',(20.6504940359422,18.3116907761807,-17.1647869918207));
#91912=CARTESIAN_POINT('Ctrl Pts',(20.647190659324,18.3046870280305,-17.1652547367467));
#91913=CARTESIAN_POINT('Ctrl Pts',(20.6456621941976,18.3014675064759,-17.1654705221608));
#91914=CARTESIAN_POINT('Ctrl Pts',(20.6421925989564,18.2942066177321,-17.1659589123766));
#91915=CARTESIAN_POINT('Ctrl Pts',(20.6402467672974,18.2901675712732,-17.1662318053479));
#91916=CARTESIAN_POINT('Ctrl Pts',(20.6344782328566,18.2782902171649,-17.1670377967522));
#91917=CARTESIAN_POINT('Ctrl Pts',(20.6306199633149,18.2704694256415,-17.1675730322893));
#91918=CARTESIAN_POINT('Ctrl Pts',(20.6028094843568,18.2149640330731,-17.171402770531));
#91919=CARTESIAN_POINT('Ctrl Pts',(20.5771121655385,18.1681802435231,-17.1747943985693));
#91920=CARTESIAN_POINT('Ctrl Pts',(20.5406293835266,18.1073293425063,-17.1793798479116));
#91921=CARTESIAN_POINT('Ctrl Pts',(20.5313932850883,18.0923508127367,-17.1805231535638));
#91922=CARTESIAN_POINT('Ctrl Pts',(20.4960017766648,18.0365251151155,-17.18483514981));
#91923=CARTESIAN_POINT('Ctrl Pts',(20.4686323362891,17.9964663709702,-17.1880325966352));
#91924=CARTESIAN_POINT('Ctrl Pts',(20.3751392973078,17.8692416741765,-17.19846191336));
#91925=CARTESIAN_POINT('Ctrl Pts',(20.3036275044895,17.7862450873941,-17.2056947123692));
#91926=CARTESIAN_POINT('Ctrl Pts',(20.1869266995004,17.6703088638426,-17.2162683604883));
#91927=CARTESIAN_POINT('Ctrl Pts',(20.1463326070025,17.6330131181074,-17.2197575867501));
#91928=CARTESIAN_POINT('Ctrl Pts',(20.0781788366405,17.5751366184986,-17.2253152820729));
#91929=CARTESIAN_POINT('Ctrl Pts',(20.0514942437143,17.5535697957619,-17.2274221920438));
#91930=CARTESIAN_POINT('Ctrl Pts',(20.0157271157714,17.5260722791464,-17.2301587689651));
#91931=CARTESIAN_POINT('Ctrl Pts',(20.0071077751816,17.519550200756,-17.230811778265));
#91932=CARTESIAN_POINT('Ctrl Pts',(19.992906284514,17.5089742805748,-17.2318772838336));
#91933=CARTESIAN_POINT('Ctrl Pts',(19.9873536792914,17.5048812646441,-17.2322913095779));
#91934=CARTESIAN_POINT('Ctrl Pts',(19.9765651487209,17.4970097606554,-17.2330908254781));
#91935=CARTESIAN_POINT('Ctrl Pts',(19.971331754115,17.4932279484552,-17.2334764419846));
#91936=CARTESIAN_POINT('Ctrl Pts',(19.9592058782948,17.4845495848669,-17.2343648594301));
#91937=CARTESIAN_POINT('Ctrl Pts',(19.9523011729783,17.4796702407674,-17.2348669943182));
#91938=CARTESIAN_POINT('Ctrl Pts',(19.9336483181675,17.466655680199,-17.2362135926313));
#91939=CARTESIAN_POINT('Ctrl Pts',(19.9218465970028,17.4585977430387,-17.23705511473));
#91940=CARTESIAN_POINT('Ctrl Pts',(19.8128219796707,17.3857657871692,-17.244736205846));
#91941=CARTESIAN_POINT('Ctrl Pts',(19.7104693969057,17.329019773098,-17.2512591646177));
#91942=CARTESIAN_POINT('Ctrl Pts',(19.4555750118391,17.2141262805561,-17.2665653516512));
#91943=CARTESIAN_POINT('Ctrl Pts',(19.300007055965,17.1645886759212,-17.2751654880419));
#91944=CARTESIAN_POINT('Ctrl Pts',(19.1084203759755,17.1271201854677,-17.2863745074836));
#91945=CARTESIAN_POINT('Ctrl Pts',(19.0763803121059,17.1216170384523,-17.2882704642959));
#91946=CARTESIAN_POINT('Ctrl Pts',(19.0370669393538,17.1157931269504,-17.2906367648735));
#91947=CARTESIAN_POINT('Ctrl Pts',(19.0299002993836,17.1147689965118,-17.2910697459533));
#91948=CARTESIAN_POINT('Ctrl Pts',(19.0186573899362,17.113221160417,-17.2917517285284));
#91949=CARTESIAN_POINT('Ctrl Pts',(19.014584530552,17.1126725207913,-17.2919993442989));
#91950=CARTESIAN_POINT('Ctrl Pts',(19.0069687910067,17.1116692023527,-17.2924634454415));
#91951=CARTESIAN_POINT('Ctrl Pts',(19.0034263488704,17.1112116295464,-17.2926797654534));
#91952=CARTESIAN_POINT('Ctrl Pts',(18.9953375040211,17.1101876096167,-17.2931747180546));
#91953=CARTESIAN_POINT('Ctrl Pts',(18.990790425775,17.109626956746,-17.2934536725306));
#91954=CARTESIAN_POINT('Ctrl Pts',(18.9768088411896,17.1079490911507,-17.2943135554647));
#91955=CARTESIAN_POINT('Ctrl Pts',(18.9673687567909,17.1068806416475,-17.2948971232507));
#91956=CARTESIAN_POINT('Ctrl Pts',(18.8825088768579,17.0978540985116,-17.3001679133913));
#91957=CARTESIAN_POINT('Ctrl Pts',(18.8067270609206,17.0938914242035,-17.3050498675469));
#91958=CARTESIAN_POINT('Ctrl Pts',(18.5459833782494,17.0942725845345,-17.3221028197883));
#91959=CARTESIAN_POINT('Ctrl Pts',(18.3618541881496,17.1187733034733,-17.3344995710412));
#91960=CARTESIAN_POINT('Ctrl Pts',(18.1318211789033,17.1807521451726,-17.3495264498624));
#91961=CARTESIAN_POINT('Ctrl Pts',(18.0809325868206,17.1965448783824,-17.3528279687531));
#91962=CARTESIAN_POINT('Ctrl Pts',(18.0188618052271,17.2184078119572,-17.3568295781235));
#91963=CARTESIAN_POINT('Ctrl Pts',(18.0070705909193,17.222679122904,-17.3575886262899));
#91964=CARTESIAN_POINT('Ctrl Pts',(17.9884944114631,17.2295955912846,-17.3587828512243));
#91965=CARTESIAN_POINT('Ctrl Pts',(17.9816840852419,17.2321713616683,-17.3592203317231));
#91966=CARTESIAN_POINT('Ctrl Pts',(17.9689419667816,17.2370659165558,-17.3600382628031));
#91967=CARTESIAN_POINT('Ctrl Pts',(17.9630071032306,17.2393764267801,-17.3604189852731));
#91968=CARTESIAN_POINT('Ctrl Pts',(17.9497498540491,17.244606639461,-17.3612689366474));
#91969=CARTESIAN_POINT('Ctrl Pts',(17.9424331431518,17.2475405393779,-17.3617376817351));
#91970=CARTESIAN_POINT('Ctrl Pts',(17.9239377700824,17.2550771167157,-17.3629218105322));
#91971=CARTESIAN_POINT('Ctrl Pts',(17.9127817374088,17.2597348422183,-17.3636353286591));
#91972=CARTESIAN_POINT('Ctrl Pts',(17.8493600421741,17.2868541353214,-17.3676884300711));
#91973=CARTESIAN_POINT('Ctrl Pts',(17.797973941112,17.3113207609099,-17.3709589032607));
#91974=CARTESIAN_POINT('Ctrl Pts',(17.7238750783338,17.3503394861406,-17.3756896543121));
#91975=CARTESIAN_POINT('Ctrl Pts',(17.7003574662086,17.3633005961775,-17.3771935453424));
#91976=CARTESIAN_POINT('Ctrl Pts',(17.5767175020271,17.4345411033099,-17.3851308845967));
#91977=CARTESIAN_POINT('Ctrl Pts',(17.481259711552,17.500517160423,-17.3913557726303));
#91978=CARTESIAN_POINT('Ctrl Pts',(17.3297861141352,17.6247218640124,-17.4020346734756));
#91979=CARTESIAN_POINT('Ctrl Pts',(17.2708275916785,17.6789362073988,-17.4064365018023));
#91980=CARTESIAN_POINT('Ctrl Pts',(17.1900064510278,17.7621835671349,-17.4130735323533));
#91981=CARTESIAN_POINT('Ctrl Pts',(17.165593140646,17.7886481760463,-17.4151676727849));
#91982=CARTESIAN_POINT('Ctrl Pts',(17.1369483323212,17.8213343243613,-17.4177541257169));
#91983=CARTESIAN_POINT('Ctrl Pts',(17.1320583903991,17.8269740627617,-17.4182003988007));
#91984=CARTESIAN_POINT('Ctrl Pts',(17.1244906025232,17.8357960891903,-17.4188987035491));
#91985=CARTESIAN_POINT('Ctrl Pts',(17.1217920799543,17.8389606715801,-17.4191492381247));
#91986=CARTESIAN_POINT('Ctrl Pts',(17.1167971617542,17.8448533402538,-17.4196158748166));
#91987=CARTESIAN_POINT('Ctrl Pts',(17.1144983275154,17.8475792842341,-17.4198317934835));
#91988=CARTESIAN_POINT('Ctrl Pts',(17.1093069381485,17.8537668570215,-17.4203220174013));
#91989=CARTESIAN_POINT('Ctrl Pts',(17.1064185682556,17.8572319135843,-17.420596620357));
#91990=CARTESIAN_POINT('Ctrl Pts',(17.0978965703123,17.8675220925263,-17.4214122651026));
#91991=CARTESIAN_POINT('Ctrl Pts',(17.0922947221149,17.8743732402815,-17.4219555195858));
#91992=CARTESIAN_POINT('Ctrl Pts',(17.0511032547075,17.9254006400831,-17.4260018821648));
#91993=CARTESIAN_POINT('Ctrl Pts',(17.0172623091447,17.9709525606907,-17.4296146850004));
#91994=CARTESIAN_POINT('Ctrl Pts',(16.9504046662844,18.0689366960563,-17.4372973740587));
#91995=CARTESIAN_POINT('Ctrl Pts',(16.9177757210432,18.121573692312,-17.4413750532935));
#91996=CARTESIAN_POINT('Ctrl Pts',(16.8338946484414,18.2711590250988,-17.4527032244226));
#91997=CARTESIAN_POINT('Ctrl Pts',(16.7877887173321,18.3707818688211,-17.4599518050173));
#91998=CARTESIAN_POINT('Ctrl Pts',(16.7481977230133,18.4773143771053,-17.4672585705686));
#91999=CARTESIAN_POINT('Ctrl Pts',(16.7468031572123,18.4811000183989,-17.467517671245));
#92000=CARTESIAN_POINT('Ctrl Pts',(16.7454194505834,18.4848895411289,-17.4677764891862));
#92001=CARTESIAN_POINT('',(16.6170006442198,19.2126515526684,-16.4878149140766));
#92002=CARTESIAN_POINT('Ctrl Pts',(16.7454194502294,18.4848895420984,-17.2426989706651));
#92003=CARTESIAN_POINT('Ctrl Pts',(16.7608133382974,18.4427306858745,-17.2398827653555));
#92004=CARTESIAN_POINT('Ctrl Pts',(16.7775450772477,18.4010690881806,-17.2371085333092));
#92005=CARTESIAN_POINT('Ctrl Pts',(16.8006203765564,18.348510109161,-17.2336175690097));
#92006=CARTESIAN_POINT('Ctrl Pts',(16.8057522413298,18.3370971610802,-17.2328600437446));
#92007=CARTESIAN_POINT('Ctrl Pts',(16.8140577699586,18.3190555931353,-17.2316632154219));
#92008=CARTESIAN_POINT('Ctrl Pts',(16.8171652140291,18.3123969747177,-17.231221645671));
#92009=CARTESIAN_POINT('Ctrl Pts',(16.8230280590362,18.300002894862,-17.2303999489647));
#92010=CARTESIAN_POINT('Ctrl Pts',(16.8257747635082,18.2942634332026,-17.2300195267569));
#92011=CARTESIAN_POINT('Ctrl Pts',(16.8319433148342,18.2815215943543,-17.2291751329545));
#92012=CARTESIAN_POINT('Ctrl Pts',(16.8353780490106,18.2745255316601,-17.2287116157621));
#92013=CARTESIAN_POINT('Ctrl Pts',(16.8455036916209,18.2541857493234,-17.2273642277309));
#92014=CARTESIAN_POINT('Ctrl Pts',(16.8522972775032,18.2408934603478,-17.2264839544724));
#92015=CARTESIAN_POINT('Ctrl Pts',(16.9092402982048,18.1323282483482,-17.2192939179738));
#92016=CARTESIAN_POINT('Ctrl Pts',(16.9664531679667,18.0409301958476,-17.2132499565895));
#92017=CARTESIAN_POINT('Ctrl Pts',(17.1097520567792,17.8466741581555,-17.1999842903702));
#92018=CARTESIAN_POINT('Ctrl Pts',(17.1991353481694,17.7468436069552,-17.1928656003642));
#92019=CARTESIAN_POINT('Ctrl Pts',(17.3093863068514,17.6449750294365,-17.1845197252994));
#92020=CARTESIAN_POINT('Ctrl Pts',(17.3215700997975,17.6339774445076,-17.1836024509762));
#92021=CARTESIAN_POINT('Ctrl Pts',(17.373685192635,17.5880246656061,-17.1796940129411));
#92022=CARTESIAN_POINT('Ctrl Pts',(17.4147922967863,17.5544386995924,-17.1766482377681));
#92023=CARTESIAN_POINT('Ctrl Pts',(17.4640563103417,17.5171854327889,-17.1729828821949));
#92024=CARTESIAN_POINT('Ctrl Pts',(17.4710311400996,17.5119783944767,-17.1724635938947));
#92025=CARTESIAN_POINT('Ctrl Pts',(17.4816439665743,17.5041568806896,-17.1716725980688));
#92026=CARTESIAN_POINT('Ctrl Pts',(17.4852585760779,17.5015106248567,-17.1714030453901));
#92027=CARTESIAN_POINT('Ctrl Pts',(17.491763703779,17.4967798610813,-17.1709176182842));
#92028=CARTESIAN_POINT('Ctrl Pts',(17.4946511079854,17.4946911630227,-17.1707020387784));
#92029=CARTESIAN_POINT('Ctrl Pts',(17.5009388108367,17.49016688858,-17.1702323249346));
#92030=CARTESIAN_POINT('Ctrl Pts',(17.5043410130771,17.4877341270827,-17.1699780083776));
#92031=CARTESIAN_POINT('Ctrl Pts',(17.5139234946811,17.4809249523921,-17.1692613162666));
#92032=CARTESIAN_POINT('Ctrl Pts',(17.5201200075639,17.4765716477264,-17.1687974061867));
#92033=CARTESIAN_POINT('Ctrl Pts',(17.5574223496223,17.4506630320028,-17.1660026203623));
#92034=CARTESIAN_POINT('Ctrl Pts',(17.5890762148143,17.4299131621867,-17.1636224139565));
#92035=CARTESIAN_POINT('Ctrl Pts',(17.6953532907791,17.3642498466803,-17.1556463338188));
#92036=CARTESIAN_POINT('Ctrl Pts',(17.7721892209598,17.3230934286936,-17.1499073692223));
#92037=CARTESIAN_POINT('Ctrl Pts',(18.0106984254139,17.2136857130653,-17.132569870025));
#92038=CARTESIAN_POINT('Ctrl Pts',(18.1785591328292,17.1606492070527,-17.1210593283118));
#92039=CARTESIAN_POINT('Ctrl Pts',(18.3736830972609,17.1247618207071,-17.1088475343449));
#92040=CARTESIAN_POINT('Ctrl Pts',(18.3963708884204,17.1209701773303,-17.107443440555));
#92041=CARTESIAN_POINT('Ctrl Pts',(18.4285581222713,17.1161287827881,-17.1054730735289));
#92042=CARTESIAN_POINT('Ctrl Pts',(18.4380091714817,17.1147725334597,-17.1048971425516));
#92043=CARTESIAN_POINT('Ctrl Pts',(18.4533813600868,17.1126726220892,-17.1039645617273));
#92044=CARTESIAN_POINT('Ctrl Pts',(18.4592969594628,17.1118899870161,-17.1036066837254));
#92045=CARTESIAN_POINT('Ctrl Pts',(18.4716873046522,17.1103040163012,-17.1028591677689));
#92046=CARTESIAN_POINT('Ctrl Pts',(18.4781626227438,17.1095055784187,-17.1024696881781));
#92047=CARTESIAN_POINT('Ctrl Pts',(18.49357731391,17.1076771758321,-17.1015452762753));
#92048=CARTESIAN_POINT('Ctrl Pts',(18.5025198127061,17.1066742416274,-17.101011201296));
#92049=CARTESIAN_POINT('Ctrl Pts',(18.5326744199962,17.1034868388343,-17.099217483476));
#92050=CARTESIAN_POINT('Ctrl Pts',(18.5539134972714,17.1015658071187,-17.0979661247632));
#92051=CARTESIAN_POINT('Ctrl Pts',(18.6697332462445,17.0928522295383,-17.091202430274));
#92052=CARTESIAN_POINT('Ctrl Pts',(18.7646647782039,17.0920986580974,-17.0858833027061));
#92053=CARTESIAN_POINT('Ctrl Pts',(19.0285280222344,17.1077480484148,-17.0713394145862));
#92054=CARTESIAN_POINT('Ctrl Pts',(19.195882176884,17.1380627443865,-17.0624207447181));
#92055=CARTESIAN_POINT('Ctrl Pts',(19.3943158318376,17.199251722985,-17.0505775159879));
#92056=CARTESIAN_POINT('Ctrl Pts',(19.4305044825888,17.2114927541701,-17.0483610744069));
#92057=CARTESIAN_POINT('Ctrl Pts',(19.473120199167,17.2272050112181,-17.0456612971868));
#92058=CARTESIAN_POINT('Ctrl Pts',(19.4798878362058,17.2297396539709,-17.0452298279612));
#92059=CARTESIAN_POINT('Ctrl Pts',(19.4908839492304,17.2339222871765,-17.0445241194717));
#92060=CARTESIAN_POINT('Ctrl Pts',(19.495120401348,17.2355493352358,-17.0442511029315));
#92061=CARTESIAN_POINT('Ctrl Pts',(19.5026782732002,17.2384799257266,-17.0437619632272));
#92062=CARTESIAN_POINT('Ctrl Pts',(19.5060016587068,17.239778254534,-17.0435461546909));
#92063=CARTESIAN_POINT('Ctrl Pts',(19.5131735701707,17.2426009850688,-17.0430788625902));
#92064=CARTESIAN_POINT('Ctrl Pts',(19.517020857971,17.2441282528494,-17.0428272125963));
#92065=CARTESIAN_POINT('Ctrl Pts',(19.5277101679921,17.2484079489913,-17.042125358408));
#92066=CARTESIAN_POINT('Ctrl Pts',(19.5345422464008,17.2511848307807,-17.0416737180217));
#92067=CARTESIAN_POINT('Ctrl Pts',(19.5733072090948,17.2671772784661,-17.0390943254087));
#92068=CARTESIAN_POINT('Ctrl Pts',(19.6049252570322,17.2811367297378,-17.0369255078848));
#92069=CARTESIAN_POINT('Ctrl Pts',(19.7038701346755,17.3277478083891,-17.0299625078815));
#92070=CARTESIAN_POINT('Ctrl Pts',(19.769812612359,17.3631965499211,-17.0250600376702));
#92071=CARTESIAN_POINT('Ctrl Pts',(19.999415570089,17.5027823087797,-17.0073370682358));
#92072=CARTESIAN_POINT('Ctrl Pts',(20.1505137405041,17.6258171798855,-16.9945246047959));
#92073=CARTESIAN_POINT('Ctrl Pts',(20.297180975354,17.7832038609921,-16.9813072130045));
#92074=CARTESIAN_POINT('Ctrl Pts',(20.3113717392771,17.7988969501502,-16.9800172853959));
#92075=CARTESIAN_POINT('Ctrl Pts',(20.3308021890409,17.8210429028221,-16.978234831391));
#92076=CARTESIAN_POINT('Ctrl Pts',(20.3362423662733,17.8273174620911,-16.9777339460917));
#92077=CARTESIAN_POINT('Ctrl Pts',(20.3455737304454,17.838208842062,-16.9768715528553));
#92078=CARTESIAN_POINT('Ctrl Pts',(20.3494823173193,17.8428105629785,-16.9765093273947));
#92079=CARTESIAN_POINT('Ctrl Pts',(20.3575399292169,17.8523797489023,-16.9757604838787));
#92080=CARTESIAN_POINT('Ctrl Pts',(20.3616859720391,17.8573496513807,-16.975373990376));
#92081=CARTESIAN_POINT('Ctrl Pts',(20.3713503100389,17.8690429902778,-16.974470263144));
#92082=CARTESIAN_POINT('Ctrl Pts',(20.3768501164111,17.8757816088079,-16.9739537837821));
#92083=CARTESIAN_POINT('Ctrl Pts',(20.394606741979,17.8978136624232,-16.9722789481775));
#92084=CARTESIAN_POINT('Ctrl Pts',(20.4066929776906,17.9132437250251,-16.9711274301937));
#92085=CARTESIAN_POINT('Ctrl Pts',(20.4676175746711,17.9932893794753,-16.9652588531404));
#92086=CARTESIAN_POINT('Ctrl Pts',(20.5129356569166,18.0605048674188,-16.9606804075939));
#92087=CARTESIAN_POINT('Ctrl Pts',(20.6403814937926,18.2751421311587,-16.9468447557961));
#92088=CARTESIAN_POINT('Ctrl Pts',(20.7088316391719,18.4298773210331,-16.9379726523065));
#92089=CARTESIAN_POINT('Ctrl Pts',(20.7740144561736,18.6427162789224,-16.9254609686511));
#92090=CARTESIAN_POINT('Ctrl Pts',(20.787845243202,18.6949340812579,-16.9223636359522));
#92091=CARTESIAN_POINT('Ctrl Pts',(20.8015778125553,18.7561511672814,-16.9186407333664));
#92092=CARTESIAN_POINT('Ctrl Pts',(20.8034390016764,18.7646955254871,-16.9181190531254));
#92093=CARTESIAN_POINT('Ctrl Pts',(20.8061752909591,18.7776425143841,-16.9173251229311));
#92094=CARTESIAN_POINT('Ctrl Pts',(20.8070894391582,18.7820369209381,-16.9170550518218));
#92095=CARTESIAN_POINT('Ctrl Pts',(20.8087044242035,18.7899260675077,-16.9165690733248));
#92096=CARTESIAN_POINT('Ctrl Pts',(20.8094104160417,18.793419697391,-16.9163534638132));
#92097=CARTESIAN_POINT('Ctrl Pts',(20.8109243812277,18.8010103023265,-16.9158841317804));
#92098=CARTESIAN_POINT('Ctrl Pts',(20.8117290458402,18.8051078358564,-16.9156302294797));
#92099=CARTESIAN_POINT('Ctrl Pts',(20.8139530056626,18.8166126562977,-16.9149158490997));
#92100=CARTESIAN_POINT('Ctrl Pts',(20.8153448309229,18.824025099657,-16.9144538520078));
#92101=CARTESIAN_POINT('Ctrl Pts',(20.8233859748052,18.8681484879154,-16.9116941377102));
#92102=CARTESIAN_POINT('Ctrl Pts',(20.8291030668226,18.9050201708442,-16.909348489043));
#92103=CARTESIAN_POINT('Ctrl Pts',(20.8446409571895,19.0263200153417,-16.9015442361564));
#92104=CARTESIAN_POINT('Ctrl Pts',(20.8503524223027,19.111187630202,-16.8959487214791));
#92105=CARTESIAN_POINT('Ctrl Pts',(20.8521980299003,19.3745107904806,-16.8785530615524));
#92106=CARTESIAN_POINT('Ctrl Pts',(20.8309048315297,19.5523405823664,-16.866831316198));
#92107=CARTESIAN_POINT('Ctrl Pts',(20.7820180809691,19.7474971384358,-16.8544506656616));
#92108=CARTESIAN_POINT('Ctrl Pts',(20.7761303999908,19.7694896887762,-16.8530611502229));
#92109=CARTESIAN_POINT('Ctrl Pts',(20.7672820275648,19.8005282998256,-16.8511075050183));
#92110=CARTESIAN_POINT('Ctrl Pts',(20.7646135002302,19.8096553576232,-16.8505339383858));
#92111=CARTESIAN_POINT('Ctrl Pts',(20.7601724701446,19.8244734254388,-16.8496041398287));
#92112=CARTESIAN_POINT('Ctrl Pts',(20.7584372914539,19.8301754005053,-16.8492466942338));
#92113=CARTESIAN_POINT('Ctrl Pts',(20.7547504591449,19.84210952208,-16.8484992507435));
#92114=CARTESIAN_POINT('Ctrl Pts',(20.7527939990759,19.8483401272186,-16.8481094148603));
#92115=CARTESIAN_POINT('Ctrl Pts',(20.7480629092415,19.8631665288297,-16.8471826438304));
#92116=CARTESIAN_POINT('Ctrl Pts',(20.74526202201,19.8717538621746,-16.8466465778249));
#92117=CARTESIAN_POINT('Ctrl Pts',(20.7356005815914,19.9007444899207,-16.8448390400018));
#92118=CARTESIAN_POINT('Ctrl Pts',(20.72848369125,19.9210614094748,-16.8435760300224));
#92119=CARTESIAN_POINT('Ctrl Pts',(20.65877648858,20.1107348947486,-16.8318107390562));
#92120=CARTESIAN_POINT('Ctrl Pts',(20.5750744889951,20.2715371396014,-16.8221162571427));
#92121=CARTESIAN_POINT('Ctrl Pts',(20.4038334576143,20.5177463402424,-16.8057909893335));
#92122=CARTESIAN_POINT('Ctrl Pts',(20.3275426677446,20.6097649082873,-16.7992390617861));
#92123=CARTESIAN_POINT('Ctrl Pts',(20.2372569729471,20.7016367454378,-16.7916051806598));
#92124=CARTESIAN_POINT('Ctrl Pts',(20.230545949909,20.7083742503944,-16.7910383510971));
#92125=CARTESIAN_POINT('Ctrl Pts',(20.2205335648251,20.718291600122,-16.7901931457129));
#92126=CARTESIAN_POINT('Ctrl Pts',(20.2172667945473,20.7215064125772,-16.7899174505304));
#92127=CARTESIAN_POINT('Ctrl Pts',(20.2114355004931,20.7272078029677,-16.7894253969436));
#92128=CARTESIAN_POINT('Ctrl Pts',(20.2088750976532,20.7296985237336,-16.7892093683627));
#92129=CARTESIAN_POINT('Ctrl Pts',(20.2033561957336,20.7350401076278,-16.7887437542423));
#92130=CARTESIAN_POINT('Ctrl Pts',(20.2003957414283,20.7378888002918,-16.7884940137176));
#92131=CARTESIAN_POINT('Ctrl Pts',(20.1921997568507,20.7457295530085,-16.7878027263656));
#92132=CARTESIAN_POINT('Ctrl Pts',(20.1869469595464,20.7507033678675,-16.7873598115959));
#92133=CARTESIAN_POINT('Ctrl Pts',(20.1580085252817,20.7778248957362,-16.7849209651063));
#92134=CARTESIAN_POINT('Ctrl Pts',(20.1338432734866,20.799451786185,-16.7828889395332));
#92135=CARTESIAN_POINT('Ctrl Pts',(19.9854221093857,20.9262650367634,-16.7704852827918));
#92136=CARTESIAN_POINT('Ctrl Pts',(19.8498706098471,21.0173842724899,-16.7595219761107));
#92137=CARTESIAN_POINT('Ctrl Pts',(19.6013597780351,21.1456932529202,-16.7412532752891));
#92138=CARTESIAN_POINT('Ctrl Pts',(19.4932263134805,21.1906298122628,-16.733807804058));
#92139=CARTESIAN_POINT('Ctrl Pts',(19.368338526942,21.2307789780287,-16.7257980463268));
#92140=CARTESIAN_POINT('Ctrl Pts',(19.3547141305646,21.2350075273089,-16.7249315762956));
#92141=CARTESIAN_POINT('Ctrl Pts',(19.3329550908196,21.2415204155779,-16.7235591941654));
#92142=CARTESIAN_POINT('Ctrl Pts',(19.3248478987339,21.2438942723837,-16.7230503667555));
#92143=CARTESIAN_POINT('Ctrl Pts',(19.3105204456,21.2479965267566,-16.7221554924122));
#92144=CARTESIAN_POINT('Ctrl Pts',(19.3043061211828,21.2497451051533,-16.7217687916749));
#92145=CARTESIAN_POINT('Ctrl Pts',(19.2914323810326,21.2533040331069,-16.7209706262376));
#92146=CARTESIAN_POINT('Ctrl Pts',(19.2847719094458,21.2551103024464,-16.7205592981371));
#92147=CARTESIAN_POINT('Ctrl Pts',(19.2676443872167,21.2596653654501,-16.7195056451325));
#92148=CARTESIAN_POINT('Ctrl Pts',(19.2571647944896,21.2623665484237,-16.718864866956));
#92149=CARTESIAN_POINT('Ctrl Pts',(19.2132694495572,21.2733226036583,-16.7161967129957));
#92150=CARTESIAN_POINT('Ctrl Pts',(19.179674500919,21.2808425458438,-16.7141930353365));
#92151=CARTESIAN_POINT('Ctrl Pts',(19.0916087532639,21.2983115691613,-16.7090282608772));
#92152=CARTESIAN_POINT('Ctrl Pts',(19.0369038015083,21.3069493188486,-16.7059069700503));
#92153=CARTESIAN_POINT('Ctrl Pts',(18.8731169370877,21.3262631490915,-16.6967386112696));
#92154=CARTESIAN_POINT('Ctrl Pts',(18.7634791437289,21.3306281634368,-16.6908401907265));
#92155=CARTESIAN_POINT('Ctrl Pts',(18.5938540381529,21.3242132902009,-16.6815973286925));
#92156=CARTESIAN_POINT('Ctrl Pts',(18.533838412007,21.3193752020727,-16.6783017826909));
#92157=CARTESIAN_POINT('Ctrl Pts',(18.4161480307497,21.3048172135664,-16.6716596722049));
#92158=CARTESIAN_POINT('Ctrl Pts',(18.3585095813221,21.2952519143196,-16.6683201738073));
#92159=CARTESIAN_POINT('Ctrl Pts',(18.292623443894,21.2814963502925,-16.6643275082868));
#92160=CARTESIAN_POINT('Ctrl Pts',(18.2839125603699,21.2796202385259,-16.6637960575681));
#92161=CARTESIAN_POINT('Ctrl Pts',(18.2707974233826,21.2767087984518,-16.6629901508239));
#92162=CARTESIAN_POINT('Ctrl Pts',(18.2663840937811,21.2757142248661,-16.6627179729499));
#92163=CARTESIAN_POINT('Ctrl Pts',(18.2584969040207,21.2739102085808,-16.662229738127));
#92164=CARTESIAN_POINT('Ctrl Pts',(18.2550218717433,21.2731061261093,-16.6620139910414));
#92165=CARTESIAN_POINT('Ctrl Pts',(18.2475085531926,21.2713476139634,-16.6615461397746));
#92166=CARTESIAN_POINT('Ctrl Pts',(18.2434710919051,21.2703901057891,-16.661293865448));
#92167=CARTESIAN_POINT('Ctrl Pts',(18.2322207231911,21.2676870521928,-16.6605885460473));
#92168=CARTESIAN_POINT('Ctrl Pts',(18.2250142226527,21.2659154600617,-16.6601340420788));
#92169=CARTESIAN_POINT('Ctrl Pts',(18.1835878735642,21.2555002336375,-16.6575063345529));
#92170=CARTESIAN_POINT('Ctrl Pts',(18.1495812600686,21.2460403221128,-16.6552902798065));
#92171=CARTESIAN_POINT('Ctrl Pts',(18.0417580379232,21.213120889428,-16.648108466777));
#92172=CARTESIAN_POINT('Ctrl Pts',(17.9689882853298,21.1864600574827,-16.6430272461827));
#92173=CARTESIAN_POINT('Ctrl Pts',(17.7276375597699,21.0826971669278,-16.6256903976212));
#92174=CARTESIAN_POINT('Ctrl Pts',(17.5677309391923,20.9874737591486,-16.6134585182406));
#92175=CARTESIAN_POINT('Ctrl Pts',(17.4027595268346,20.8572395274554,-16.6004980487838));
#92176=CARTESIAN_POINT('Ctrl Pts',(17.3835382494091,20.8415087922951,-16.5989801576873));
#92177=CARTESIAN_POINT('Ctrl Pts',(17.3570805703094,20.8190668653724,-16.5968788920727));
#92178=CARTESIAN_POINT('Ctrl Pts',(17.3496081024696,20.8126382982942,-16.5962840607804));
#92179=CARTESIAN_POINT('Ctrl Pts',(17.3376414850434,20.8021970929332,-16.5953291730991));
#92180=CARTESIAN_POINT('Ctrl Pts',(17.3331191541901,20.7982171079787,-16.5949677708059));
#92181=CARTESIAN_POINT('Ctrl Pts',(17.3240601040195,20.7901755969321,-16.5942426998683));
#92182=CARTESIAN_POINT('Ctrl Pts',(17.3195237958012,20.7861136927771,-16.5938790520863));
#92183=CARTESIAN_POINT('Ctrl Pts',(17.308815303024,20.7764415187106,-16.5930192243498));
#92184=CARTESIAN_POINT('Ctrl Pts',(17.3026585954686,20.7708142055097,-16.5925237697993));
#92185=CARTESIAN_POINT('Ctrl Pts',(17.2835087793866,20.7531021601161,-16.5909790765961));
#92186=CARTESIAN_POINT('Ctrl Pts',(17.2706340332799,20.7408901689957,-16.589935275857));
#92187=CARTESIAN_POINT('Ctrl Pts',(17.2410163613195,20.7120811236827,-16.587520381117));
#92188=CARTESIAN_POINT('Ctrl Pts',(17.2243939338661,20.6953632550145,-16.5861545741598));
#92189=CARTESIAN_POINT('Ctrl Pts',(17.1679487870902,20.636664891547,-16.5814744621242));
#92190=CARTESIAN_POINT('Ctrl Pts',(17.1295686553656,20.5933304868224,-16.5782181253249));
#92191=CARTESIAN_POINT('Ctrl Pts',(16.9902367712116,20.4223798814947,-16.5659819735331));
#92192=CARTESIAN_POINT('Ctrl Pts',(16.9023477456282,20.2848695605904,-16.5574009865093));
#92193=CARTESIAN_POINT('Ctrl Pts',(16.8040977614397,20.0833278367252,-16.5448725997813));
#92194=CARTESIAN_POINT('Ctrl Pts',(16.779551817381,20.0268488270614,-16.541360640526));
#92195=CARTESIAN_POINT('Ctrl Pts',(16.754233554344,19.9608647474203,-16.5371690538814));
#92196=CARTESIAN_POINT('Ctrl Pts',(16.7510188204722,19.9523217612051,-16.5366246936974));
#92197=CARTESIAN_POINT('Ctrl Pts',(16.7462992686397,19.9395294237985,-16.5358066925635));
#92198=CARTESIAN_POINT('Ctrl Pts',(16.7447525651962,19.9352954929125,-16.5355354877355));
#92199=CARTESIAN_POINT('Ctrl Pts',(16.7420066161964,19.9277036158188,-16.5350482980861));
#92200=CARTESIAN_POINT('Ctrl Pts',(16.7408023220002,19.9243475521669,-16.5348326175953));
#92201=CARTESIAN_POINT('Ctrl Pts',(16.7382108441443,19.9170679593546,-16.5343640962465));
#92202=CARTESIAN_POINT('Ctrl Pts',(16.7368267677674,19.9131434309484,-16.5341110808477));
#92203=CARTESIAN_POINT('Ctrl Pts',(16.7329885652896,19.9021570952751,-16.5334016414113));
#92204=CARTESIAN_POINT('Ctrl Pts',(16.7305602908146,19.8950864126831,-16.5329437312795));
#92205=CARTESIAN_POINT('Ctrl Pts',(16.7165951444969,19.8537103629048,-16.5302570475579));
#92206=CARTESIAN_POINT('Ctrl Pts',(16.7059028430342,19.8191287041954,-16.5279831894366));
#92207=CARTESIAN_POINT('Ctrl Pts',(16.6742359297377,19.7065615433117,-16.5205278820005));
#92208=CARTESIAN_POINT('Ctrl Pts',(16.6568356156139,19.6276481163896,-16.5152217318738));
#92209=CARTESIAN_POINT('Ctrl Pts',(16.62611250444,19.4370747924495,-16.502476141204));
#92210=CARTESIAN_POINT('Ctrl Pts',(16.6170882586042,19.3249577472053,-16.4950407472082));
#92211=CARTESIAN_POINT('Ctrl Pts',(16.6170006442198,19.2126515526684,-16.4878149140766));
#92212=CARTESIAN_POINT('Ctrl Pts',(16.6170006421843,19.2126489414195,-16.4878147460677));
#92213=CARTESIAN_POINT('Ctrl Pts',(16.6169350225893,19.1284029889612,-16.4823943244624));
#92214=CARTESIAN_POINT('Ctrl Pts',(16.6218981987403,19.0442181697761,-16.4770994291474));
#92215=CARTESIAN_POINT('Ctrl Pts',(16.633098807133,18.950209986943,-16.471327040016));
#92216=CARTESIAN_POINT('Ctrl Pts',(16.6344059066889,18.9398876570459,-16.4706950623719));
#92217=CARTESIAN_POINT('Ctrl Pts',(16.6367383501716,18.9224977218493,-16.4696333979581));
#92218=CARTESIAN_POINT('Ctrl Pts',(16.6377234420822,18.9154249891837,-16.4692024488237));
#92219=CARTESIAN_POINT('Ctrl Pts',(16.6396009380811,18.9024267101138,-16.468411965802));
#92220=CARTESIAN_POINT('Ctrl Pts',(16.6404827474481,18.8964997293883,-16.4680521005657));
#92221=CARTESIAN_POINT('Ctrl Pts',(16.6423536700329,18.8842811744395,-16.467311403041));
#92222=CARTESIAN_POINT('Ctrl Pts',(16.6433460343017,18.8779901537177,-16.4669306778651));
#92223=CARTESIAN_POINT('Ctrl Pts',(16.6456303028101,18.8639219699515,-16.4660806816276));
#92224=CARTESIAN_POINT('Ctrl Pts',(16.6469372952589,18.8561473261561,-16.4656118946186));
#92225=CARTESIAN_POINT('Ctrl Pts',(16.6503588008126,18.836467557097,-16.4644275879081));
#92226=CARTESIAN_POINT('Ctrl Pts',(16.6525319517277,18.8245728129953,-16.4637139347788));
#92227=CARTESIAN_POINT('Ctrl Pts',(16.6655166178299,18.7567911540029,-16.4596586380029));
#92228=CARTESIAN_POINT('Ctrl Pts',(16.6784773403236,18.701336772074,-16.456386194377));
#92229=CARTESIAN_POINT('Ctrl Pts',(16.7044778881151,18.6073650743949,-16.4508783799238));
#92230=CARTESIAN_POINT('Ctrl Pts',(16.7164194104933,18.568579643663,-16.4486161308946));
#92231=CARTESIAN_POINT('Ctrl Pts',(16.7346150747456,18.5150079072523,-16.4454901792472));
#92232=CARTESIAN_POINT('Ctrl Pts',(16.7399323961956,18.4999168000981,-16.4446094297424));
#92233=CARTESIAN_POINT('Ctrl Pts',(16.7454194446555,18.4848895573635,-16.4437313838642));
#92234=CARTESIAN_POINT('Origin',(18.734,19.211,0.));
#92235=CARTESIAN_POINT('',(16.7454194503191,18.4848895418527,-15.6464962064494));
#92236=CARTESIAN_POINT('',(16.7454194505387,18.4848895412514,-15.8662164192772));
#92237=CARTESIAN_POINT('',(16.7454194503191,18.4848895418526,0.));
#92238=CARTESIAN_POINT('Ctrl Pts',(16.7454194505387,18.4848895412513,-15.8662164192772));
#92239=CARTESIAN_POINT('Ctrl Pts',(16.7372703379848,18.5072073119498,-15.8675066544822));
#92240=CARTESIAN_POINT('Ctrl Pts',(16.7294937210257,18.5296710612778,-15.8687971937546));
#92241=CARTESIAN_POINT('Ctrl Pts',(16.6950140122692,18.6349799328782,-15.8748264215078));
#92242=CARTESIAN_POINT('Ctrl Pts',(16.6730620585041,18.7192730630267,-15.879590771347));
#92243=CARTESIAN_POINT('Ctrl Pts',(16.6490998728355,18.8417960952826,-15.8867186438287));
#92244=CARTESIAN_POINT('Ctrl Pts',(16.6428359561586,18.8791075386946,-15.8889160378287));
#92245=CARTESIAN_POINT('Ctrl Pts',(16.6365221776738,18.9240625137794,-15.8916169870224));
#92246=CARTESIAN_POINT('Ctrl Pts',(16.6355092984658,18.9315664519105,-15.8920696099598));
#92247=CARTESIAN_POINT('Ctrl Pts',(16.6339995009993,18.9432232343556,-15.8927757052441));
#92248=CARTESIAN_POINT('Ctrl Pts',(16.6334745846743,18.9473724769717,-15.8930276259775));
#92249=CARTESIAN_POINT('Ctrl Pts',(16.6325251662833,18.955060116845,-15.8934955089828));
#92250=CARTESIAN_POINT('Ctrl Pts',(16.6320973022233,18.9585980407536,-15.8937112793496));
#92251=CARTESIAN_POINT('Ctrl Pts',(16.6311517265414,18.9665859877452,-15.8941994496842));
#92252=CARTESIAN_POINT('Ctrl Pts',(16.6306392092088,18.9710365580287,-15.8944721366715));
#92253=CARTESIAN_POINT('Ctrl Pts',(16.6291723812532,18.9841399594694,-15.8952769688769));
#92254=CARTESIAN_POINT('Ctrl Pts',(16.6282573251072,18.992796966599,-15.8958112422079));
#92255=CARTESIAN_POINT('Ctrl Pts',(16.6221408152905,19.0542888849057,-15.8996231389614));
#92256=CARTESIAN_POINT('Ctrl Pts',(16.6188755553195,19.1072929604781,-15.9029969137695));
#92257=CARTESIAN_POINT('Ctrl Pts',(16.6172125016239,19.1767948315625,-15.9074892765317));
#92258=CARTESIAN_POINT('Ctrl Pts',(16.6170107019972,19.1932348624198,-15.9085569473233));
#92259=CARTESIAN_POINT('Ctrl Pts',(16.6169886661989,19.2284497820847,-15.9108526786612));
#92260=CARTESIAN_POINT('Ctrl Pts',(16.6172266699904,19.2472233291539,-15.9120818925368));
#92261=CARTESIAN_POINT('Ctrl Pts',(16.6217705396517,19.4220908626881,-15.9235687497658));
#92262=CARTESIAN_POINT('Ctrl Pts',(16.6430867859052,19.5772852807938,-15.9339905157257));
#92263=CARTESIAN_POINT('Ctrl Pts',(16.6824567722274,19.7333814825322,-15.9442508721972));
#92264=CARTESIAN_POINT('Ctrl Pts',(16.6836461856932,19.7380306114362,-15.9445563049051));
#92265=CARTESIAN_POINT('Ctrl Pts',(16.700756637075,19.8039765604478,-15.9488864316136));
#92266=CARTESIAN_POINT('Ctrl Pts',(16.7194057233029,19.8645372993343,-15.9528331057524));
#92267=CARTESIAN_POINT('Ctrl Pts',(16.744959207958,19.935956743936,-15.9574536552498));
#92268=CARTESIAN_POINT('Ctrl Pts',(16.7492787226897,19.9477000847883,-15.958212341309));
#92269=CARTESIAN_POINT('Ctrl Pts',(16.756535005512,19.966900394793,-15.9594512072949));
#92270=CARTESIAN_POINT('Ctrl Pts',(16.7594104063373,19.974380082677,-15.9599334245396));
#92271=CARTESIAN_POINT('Ctrl Pts',(16.7646512558223,19.9877851863247,-15.9607969988478));
#92272=CARTESIAN_POINT('Ctrl Pts',(16.7670011407485,19.9937165457377,-15.9611788728995));
#92273=CARTESIAN_POINT('Ctrl Pts',(16.7720573989489,20.0063124979173,-15.9619893728709));
#92274=CARTESIAN_POINT('Ctrl Pts',(16.7747710038254,20.0129741153373,-15.9624177491541));
#92275=CARTESIAN_POINT('Ctrl Pts',(16.7821562834052,20.0308429904551,-15.9635661535161));
#92276=CARTESIAN_POINT('Ctrl Pts',(16.7868905535818,20.042024208996,-15.9642840543624));
#92277=CARTESIAN_POINT('Ctrl Pts',(16.8108460052971,20.0972725461428,-15.9678286378448));
#92278=CARTESIAN_POINT('Ctrl Pts',(16.8314690797192,20.1407187370143,-15.9706070439605));
#92279=CARTESIAN_POINT('Ctrl Pts',(16.9305671038933,20.3323508844003,-15.9828817081904));
#92280=CARTESIAN_POINT('Ctrl Pts',(17.0249934829181,20.4715936178588,-15.9917999865555));
#92281=CARTESIAN_POINT('Ctrl Pts',(17.1995485361948,20.6728115048001,-16.0063839212129));
#92282=CARTESIAN_POINT('Ctrl Pts',(17.2693654620147,20.7427554364548,-16.0118766883602));
#92283=CARTESIAN_POINT('Ctrl Pts',(17.3511068413779,20.8139315351939,-16.0182979628849));
#92284=CARTESIAN_POINT('Ctrl Pts',(17.3584620166462,20.8202477257904,-16.0188757012464));
#92285=CARTESIAN_POINT('Ctrl Pts',(17.3693853964042,20.829498478165,-16.0197340841584));
#92286=CARTESIAN_POINT('Ctrl Pts',(17.3729203592993,20.8324723404708,-16.0200119253745));
#92287=CARTESIAN_POINT('Ctrl Pts',(17.379208746065,20.8377275260725,-16.0205063378721));
#92288=CARTESIAN_POINT('Ctrl Pts',(17.3819582459753,20.8400134686323,-16.0207225671721));
#92289=CARTESIAN_POINT('Ctrl Pts',(17.3878614411671,20.8448961621785,-16.0211869480593));
#92290=CARTESIAN_POINT('Ctrl Pts',(17.3910168175665,20.847490714733,-16.0214352458989));
#92291=CARTESIAN_POINT('Ctrl Pts',(17.399698556077,20.8545873772714,-16.0221185784219));
#92292=CARTESIAN_POINT('Ctrl Pts',(17.405240118824,20.8590706856279,-16.0225549306345));
#92293=CARTESIAN_POINT('Ctrl Pts',(17.4349422088294,20.8828534803047,-16.0248941948067));
#92294=CARTESIAN_POINT('Ctrl Pts',(17.4594994325259,20.9016487733083,-16.0268298793207));
#92295=CARTESIAN_POINT('Ctrl Pts',(17.5350662576103,20.9569030432717,-16.032769249948));
#92296=CARTESIAN_POINT('Ctrl Pts',(17.5872901051328,20.991638894754,-16.0368503662621));
#92297=CARTESIAN_POINT('Ctrl Pts',(17.7561738807176,21.0934557490769,-16.0498093867847));
#92298=CARTESIAN_POINT('Ctrl Pts',(17.8777424423705,21.1517760712222,-16.0587750403475));
#92299=CARTESIAN_POINT('Ctrl Pts',(18.0423576948902,21.2122464713815,-16.0700684915993));
#92300=CARTESIAN_POINT('Ctrl Pts',(18.0810896173937,21.2252156957783,-16.0726704383924));
#92301=CARTESIAN_POINT('Ctrl Pts',(18.1665838700041,21.2511175143233,-16.0782894123099));
#92302=CARTESIAN_POINT('Ctrl Pts',(18.2134654325085,21.26358006063,-16.0812910215525));
#92303=CARTESIAN_POINT('Ctrl Pts',(18.2730119900446,21.2772375612181,-16.0850068878458));
#92304=CARTESIAN_POINT('Ctrl Pts',(18.2853121770729,21.2799434146481,-16.0857693559484));
#92305=CARTESIAN_POINT('Ctrl Pts',(18.3048443108914,21.2840578043013,-16.0869722262839));
#92306=CARTESIAN_POINT('Ctrl Pts',(18.3120605779536,21.28553859731,-16.0874149339052));
#92307=CARTESIAN_POINT('Ctrl Pts',(18.3255227062038,21.2882279048498,-16.0882376989306));
#92308=CARTESIAN_POINT('Ctrl Pts',(18.3317665506242,21.2894459872229,-16.0886180580254));
#92309=CARTESIAN_POINT('Ctrl Pts',(18.3456487794615,21.2920893069624,-16.0894610037054));
#92310=CARTESIAN_POINT('Ctrl Pts',(18.3532897352393,21.2935006772667,-16.0899231436532));
#92311=CARTESIAN_POINT('Ctrl Pts',(18.3755207990142,21.2974805594587,-16.09126252262));
#92312=CARTESIAN_POINT('Ctrl Pts',(18.390130499251,21.2999380665025,-16.0921362302239));
#92313=CARTESIAN_POINT('Ctrl Pts',(18.5067618485589,21.3182999358133,-16.0990618573236));
#92314=CARTESIAN_POINT('Ctrl Pts',(18.6098034071758,21.32687556893,-16.1048707490221));
#92315=CARTESIAN_POINT('Ctrl Pts',(18.8727090876753,21.3294748362667,-16.1193461025518));
#92316=CARTESIAN_POINT('Ctrl Pts',(19.0319979647193,21.3129907613249,-16.1277744772072));
#92317=CARTESIAN_POINT('Ctrl Pts',(19.2353151291203,21.2683594659664,-16.1395295669706));
#92318=CARTESIAN_POINT('Ctrl Pts',(19.2823474315499,21.2563261688315,-16.142324317089));
#92319=CARTESIAN_POINT('Ctrl Pts',(19.3363663344937,21.2405083128188,-16.1456660095503));
#92320=CARTESIAN_POINT('Ctrl Pts',(19.3437999112581,21.2382871668293,-16.1461287968799));
#92321=CARTESIAN_POINT('Ctrl Pts',(19.3556667038689,21.2346702077863,-16.1468725286104));
#92322=CARTESIAN_POINT('Ctrl Pts',(19.3601079030015,21.2333005447848,-16.1471519859625));
#92323=CARTESIAN_POINT('Ctrl Pts',(19.3679699771556,21.2308475051833,-16.1476487304446));
#92324=CARTESIAN_POINT('Ctrl Pts',(19.3713926503351,21.2297700426906,-16.1478656690635));
#92325=CARTESIAN_POINT('Ctrl Pts',(19.3786461899969,21.2274663320713,-16.1483268959632));
#92326=CARTESIAN_POINT('Ctrl Pts',(19.3824762460304,21.2262378858005,-16.1485713065385));
#92327=CARTESIAN_POINT('Ctrl Pts',(19.3928140280941,21.2228896393008,-16.1492333101437));
#92328=CARTESIAN_POINT('Ctrl Pts',(19.3993149475863,21.2207492037316,-16.1496520895752));
#92329=CARTESIAN_POINT('Ctrl Pts',(19.4316549186143,21.2099271234083,-16.1517473445269));
#92330=CARTESIAN_POINT('Ctrl Pts',(19.4573336978648,21.200778939605,-16.1534491572841));
#92331=CARTESIAN_POINT('Ctrl Pts',(19.5312492754909,21.1728263444362,-16.158444594095));
#92332=CARTESIAN_POINT('Ctrl Pts',(19.5789802184669,21.1527457923717,-16.1617914264722));
#92333=CARTESIAN_POINT('Ctrl Pts',(19.7513291389154,21.0726795994349,-16.1742136793461));
#92334=CARTESIAN_POINT('Ctrl Pts',(19.8707357306342,21.0022692271514,-16.183460321891));
#92335=CARTESIAN_POINT('Ctrl Pts',(20.0600503310996,20.8640331959325,-16.1986385612822));
#92336=CARTESIAN_POINT('Ctrl Pts',(20.1337362630978,20.802122586771,-16.204711127236));
#92337=CARTESIAN_POINT('Ctrl Pts',(20.2129594146628,20.7257807064029,-16.2114253132841));
#92338=CARTESIAN_POINT('Ctrl Pts',(20.2228563979325,20.716054211461,-16.2122678391311));
#92339=CARTESIAN_POINT('Ctrl Pts',(20.2385435219477,20.7003311406643,-16.2136095515018));
#92340=CARTESIAN_POINT('Ctrl Pts',(20.2443949946132,20.6943965819486,-16.2141114538958));
#92341=CARTESIAN_POINT('Ctrl Pts',(20.2547040314954,20.6838169237359,-16.2149983082703));
#92342=CARTESIAN_POINT('Ctrl Pts',(20.259175711001,20.6791857832855,-16.2153838770409));
#92343=CARTESIAN_POINT('Ctrl Pts',(20.2684305518141,20.6695130017695,-16.2161837577181));
#92344=CARTESIAN_POINT('Ctrl Pts',(20.2732101580416,20.6644680546276,-16.2165979129536));
#92345=CARTESIAN_POINT('Ctrl Pts',(20.2855195851536,20.6513464527358,-16.2176673607829));
#92346=CARTESIAN_POINT('Ctrl Pts',(20.2930112736187,20.6432341927009,-16.2183210147964));
#92347=CARTESIAN_POINT('Ctrl Pts',(20.3249209678904,20.608134216241,-16.221117670866));
#92348=CARTESIAN_POINT('Ctrl Pts',(20.3487051625018,20.5805769477522,-16.2232339635939));
#92349=CARTESIAN_POINT('Ctrl Pts',(20.4096666454325,20.5061477177143,-16.2287591338815));
#92350=CARTESIAN_POINT('Ctrl Pts',(20.4455890093664,20.4582891297163,-16.2321205143551));
#92351=CARTESIAN_POINT('Ctrl Pts',(20.5743805507534,20.2706403478866,-16.2447295331557));
#92352=CARTESIAN_POINT('Ctrl Pts',(20.6525332045611,20.1215278360038,-16.2535600900867));
#92353=CARTESIAN_POINT('Ctrl Pts',(20.7314606050521,19.9143827251244,-16.2660207074756));
#92354=CARTESIAN_POINT('Ctrl Pts',(20.748724706781,19.8632878456706,-16.2691133167137));
#92355=CARTESIAN_POINT('Ctrl Pts',(20.7664984018001,19.803212511083,-16.2728309609752));
#92356=CARTESIAN_POINT('Ctrl Pts',(20.768926347849,19.7948151800642,-16.273352439142));
#92357=CARTESIAN_POINT('Ctrl Pts',(20.772521955724,19.7820843862449,-16.2741461215025));
#92358=CARTESIAN_POINT('Ctrl Pts',(20.7737279911564,19.7777617324963,-16.2744161488845));
#92359=CARTESIAN_POINT('Ctrl Pts',(20.7758672021795,19.7699991348371,-16.2749020808522));
#92360=CARTESIAN_POINT('Ctrl Pts',(20.7768054426064,19.7665606424587,-16.2751176878113));
#92361=CARTESIAN_POINT('Ctrl Pts',(20.7788242211849,19.7590879005226,-16.2755870519059));
#92362=CARTESIAN_POINT('Ctrl Pts',(20.7799014919576,19.7550528712854,-16.275840989026));
#92363=CARTESIAN_POINT('Ctrl Pts',(20.782891330925,19.7437196596552,-16.2765555634833));
#92364=CARTESIAN_POINT('Ctrl Pts',(20.7847768123271,19.7364144876266,-16.277017721132));
#92365=CARTESIAN_POINT('Ctrl Pts',(20.7957646678839,19.6928824517357,-16.2797803557153));
#92366=CARTESIAN_POINT('Ctrl Pts',(20.8039453947512,19.656432273043,-16.2821288798174));
#92367=CARTESIAN_POINT('Ctrl Pts',(20.8276015321951,19.5362292035531,-16.2899473316017));
#92368=CARTESIAN_POINT('Ctrl Pts',(20.8389879282697,19.4517599740834,-16.2955546762976));
#92369=CARTESIAN_POINT('Ctrl Pts',(20.8583669163958,19.1892229037362,-16.3129454354005));
#92370=CARTESIAN_POINT('Ctrl Pts',(20.8490135372426,19.0106221892133,-16.3246495988053));
#92371=CARTESIAN_POINT('Ctrl Pts',(20.8133485376991,18.8128570185984,-16.3370162763271));
#92372=CARTESIAN_POINT('Ctrl Pts',(20.8089427716754,18.7904994258932,-16.3384070634925));
#92373=CARTESIAN_POINT('Ctrl Pts',(20.802187213201,18.7589146812718,-16.3403621679231));
#92374=CARTESIAN_POINT('Ctrl Pts',(20.8001349567033,18.7496261498893,-16.3409359412275));
#92375=CARTESIAN_POINT('Ctrl Pts',(20.7966949663175,18.7345401321159,-16.3418659829541));
#92376=CARTESIAN_POINT('Ctrl Pts',(20.7953452462647,18.7287341950681,-16.3422234663102));
#92377=CARTESIAN_POINT('Ctrl Pts',(20.7924655646804,18.7165799772789,-16.3429709157617));
#92378=CARTESIAN_POINT('Ctrl Pts',(20.790930714254,18.7102329103519,-16.3433607201655));
#92379=CARTESIAN_POINT('Ctrl Pts',(20.7872036082603,18.6951264955355,-16.3442872831915));
#92380=CARTESIAN_POINT('Ctrl Pts',(20.7849846198863,18.6863738260265,-16.3448231737148));
#92381=CARTESIAN_POINT('Ctrl Pts',(20.7772909391374,18.6568215804738,-16.3466294900107));
#92382=CARTESIAN_POINT('Ctrl Pts',(20.7715551903311,18.6360908948829,-16.3478914697358));
#92383=CARTESIAN_POINT('Ctrl Pts',(20.7148905508003,18.4427996760088,-16.3596190630719));
#92384=CARTESIAN_POINT('Ctrl Pts',(20.6424768867629,18.2773073149672,-16.3692832525787));
#92385=CARTESIAN_POINT('Ctrl Pts',(20.4883295364103,18.0200282347763,-16.3856074761936));
#92386=CARTESIAN_POINT('Ctrl Pts',(20.4180311589327,17.9225449017254,-16.3921923595659));
#92387=CARTESIAN_POINT('Ctrl Pts',(20.3336713427506,17.8243381489574,-16.3998650207705));
#92388=CARTESIAN_POINT('Ctrl Pts',(20.3274243060859,17.8171641175908,-16.4004320371321));
#92389=CARTESIAN_POINT('Ctrl Pts',(20.3180957235876,17.8065959444037,-16.4012774683594));
#92390=CARTESIAN_POINT('Ctrl Pts',(20.3150510616812,17.8031692032372,-16.4015532005077));
#92391=CARTESIAN_POINT('Ctrl Pts',(20.3096140319301,17.7970897543647,-16.4020452945855));
#92392=CARTESIAN_POINT('Ctrl Pts',(20.3072260558671,17.7944331864542,-16.4022613264826));
#92393=CARTESIAN_POINT('Ctrl Pts',(20.3020773230243,17.7887344181768,-16.4027269186725));
#92394=CARTESIAN_POINT('Ctrl Pts',(20.2993144721353,17.7856942507366,-16.4029766337973));
#92395=CARTESIAN_POINT('Ctrl Pts',(20.2916632600421,17.7773241394906,-16.4036677807611));
#92396=CARTESIAN_POINT('Ctrl Pts',(20.2867564615553,17.7720112327354,-16.4041105796447));
#92397=CARTESIAN_POINT('Ctrl Pts',(20.2597183887548,17.7430346861219,-16.406547622935));
#92398=CARTESIAN_POINT('Ctrl Pts',(20.2370746040844,17.719857742163,-16.4085778995664));
#92399=CARTESIAN_POINT('Ctrl Pts',(20.097483666602,17.5833909361846,-16.4209809736149));
#92400=CARTESIAN_POINT('Ctrl Pts',(19.9683196361249,17.483384903518,-16.431945889431));
#92401=CARTESIAN_POINT('Ctrl Pts',(19.7289717787905,17.3387359982418,-16.4502134574942));
#92402=CARTESIAN_POINT('Ctrl Pts',(19.6241279329738,17.2866763765054,-16.4576564236641));
#92403=CARTESIAN_POINT('Ctrl Pts',(19.502224009768,17.2382544165585,-16.4656656123793));
#92404=CARTESIAN_POINT('Ctrl Pts',(19.4888880039725,17.233112899239,-16.4665337624093));
#92405=CARTESIAN_POINT('Ctrl Pts',(19.4675809827548,17.2251451628107,-16.4679082935556));
#92406=CARTESIAN_POINT('Ctrl Pts',(19.4596435150015,17.2222310377965,-16.4684176042152));
#92407=CARTESIAN_POINT('Ctrl Pts',(19.4456142188266,17.2171755607581,-16.4693130406014));
#92408=CARTESIAN_POINT('Ctrl Pts',(19.4395296934197,17.2150143928148,-16.4696998227235));
#92409=CARTESIAN_POINT('Ctrl Pts',(19.4269249419875,17.2106021387253,-16.4704978804469));
#92410=CARTESIAN_POINT('Ctrl Pts',(19.420403403652,17.2083550120386,-16.470909020808));
#92411=CARTESIAN_POINT('Ctrl Pts',(19.4036362681259,17.2026690853815,-16.4719616220111));
#92412=CARTESIAN_POINT('Ctrl Pts',(19.3933750308138,17.1992767661786,-16.472601542176));
#92413=CARTESIAN_POINT('Ctrl Pts',(19.3504478183054,17.1854489578652,-16.4752613457933));
#92414=CARTESIAN_POINT('Ctrl Pts',(19.3175556178848,17.1757290170095,-16.4772577199586));
#92415=CARTESIAN_POINT('Ctrl Pts',(19.2312587993225,17.1524917941883,-16.4823994168371));
#92416=CARTESIAN_POINT('Ctrl Pts',(19.1775362635816,17.1402516873574,-16.4855053983549));
#92417=CARTESIAN_POINT('Ctrl Pts',(19.0159374463888,17.1100117523139,-16.4946470567729));
#92418=CARTESIAN_POINT('Ctrl Pts',(18.9070813659006,17.0982567435247,-16.5005339951662));
#92419=CARTESIAN_POINT('Ctrl Pts',(18.7545609007622,17.0936578019592,-16.5088415043364));
#92420=CARTESIAN_POINT('Ctrl Pts',(18.7112882878485,17.0936798263302,-16.511206511981));
#92421=CARTESIAN_POINT('Ctrl Pts',(18.5928088297098,17.0973726713773,-16.5177696490504));
#92422=CARTESIAN_POINT('Ctrl Pts',(18.5177564429834,17.1037288720893,-16.5220238639938));
#92423=CARTESIAN_POINT('Ctrl Pts',(18.4338140958387,17.1153694449363,-16.527046513207));
#92424=CARTESIAN_POINT('Ctrl Pts',(18.4244262290748,17.1167356725686,-16.5276120009833));
#92425=CARTESIAN_POINT('Ctrl Pts',(18.410521447902,17.1188547869544,-16.5284555842056));
#92426=CARTESIAN_POINT('Ctrl Pts',(18.4059971338908,17.1195593278658,-16.5287310139246));
#92427=CARTESIAN_POINT('Ctrl Pts',(18.3979478499815,17.1208395493804,-16.5292227772194));
#92428=CARTESIAN_POINT('Ctrl Pts',(18.3944220163879,17.1214094779884,-16.529438782477));
#92429=CARTESIAN_POINT('Ctrl Pts',(18.3868404970197,17.1226546780927,-16.5299045559549));
#92430=CARTESIAN_POINT('Ctrl Pts',(18.3827853905457,17.1233328326854,-16.5301544802672));
#92431=CARTESIAN_POINT('Ctrl Pts',(18.371587516295,17.1252390551038,-16.5308467825892));
#92432=CARTESIAN_POINT('Ctrl Pts',(18.3644491185967,17.1264919836675,-16.5312905350325));
#92433=CARTESIAN_POINT('Ctrl Pts',(18.3252126943376,17.1335866200963,-16.5337424573576));
#92434=CARTESIAN_POINT('Ctrl Pts',(18.2932484482161,17.140132739488,-16.5357871695786));
#92435=CARTESIAN_POINT('Ctrl Pts',(18.1029248986742,17.1837157752577,-16.5481950996584));
#92436=CARTESIAN_POINT('Ctrl Pts',(17.9491147409275,17.2381613894483,-16.5591467914266));
#92437=CARTESIAN_POINT('Ctrl Pts',(17.6981779518302,17.3610276539101,-16.5773969661328));
#92438=CARTESIAN_POINT('Ctrl Pts',(17.5977168659777,17.4209739011093,-16.5848353107958));
#92439=CARTESIAN_POINT('Ctrl Pts',(17.4910707273739,17.4972263303822,-16.5928404804345));
#92440=CARTESIAN_POINT('Ctrl Pts',(17.4795260830902,17.5056588098105,-16.5937088485083));
#92441=CARTESIAN_POINT('Ctrl Pts',(17.4612896757661,17.5192645181367,-16.5950836585368));
#92442=CARTESIAN_POINT('Ctrl Pts',(17.4545421215723,17.5243619088323,-16.5955930318842));
#92443=CARTESIAN_POINT('Ctrl Pts',(17.4426965018002,17.5334225893669,-16.596488541193));
#92444=CARTESIAN_POINT('Ctrl Pts',(17.4375857206993,17.5373690039356,-16.5968753338861));
#92445=CARTESIAN_POINT('Ctrl Pts',(17.4272245941441,17.5454455395872,-16.5976603896072));
#92446=CARTESIAN_POINT('Ctrl Pts',(17.4219755787544,17.5495772538036,-16.5980585832868));
#92447=CARTESIAN_POINT('Ctrl Pts',(17.4086671173706,17.5601552898741,-16.5990694540297));
#92448=CARTESIAN_POINT('Ctrl Pts',(17.4006350326858,17.5666358747579,-16.5996807535804));
#92449=CARTESIAN_POINT('Ctrl Pts',(17.3833150855723,17.5808206026031,-16.601001764251));
#92450=CARTESIAN_POINT('Ctrl Pts',(17.3740450221823,17.5885459719998,-16.6017106003301));
#92451=CARTESIAN_POINT('Ctrl Pts',(17.3475939486691,17.6109754286509,-16.6037388864044));
#92452=CARTESIAN_POINT('Ctrl Pts',(17.3305815226943,17.6258763451671,-16.6050504124132));
#92453=CARTESIAN_POINT('Ctrl Pts',(17.2733864286901,17.6776154003413,-16.6094885510654));
#92454=CARTESIAN_POINT('Ctrl Pts',(17.234387828678,17.7157326999588,-16.6125639121214));
#92455=CARTESIAN_POINT('Ctrl Pts',(17.1220538387575,17.8343492803952,-16.6216520988581));
#92456=CARTESIAN_POINT('Ctrl Pts',(17.0534108180664,17.9190408009899,-16.6275160212359));
#92457=CARTESIAN_POINT('Ctrl Pts',(16.9234840446183,18.1073250390856,-16.6399672490605));
#92458=CARTESIAN_POINT('Ctrl Pts',(16.8638998449213,18.2116084425544,-16.6465480196933));
#92459=CARTESIAN_POINT('Ctrl Pts',(16.8094654166003,18.3289874233287,-16.6542160118183));
#92460=CARTESIAN_POINT('Ctrl Pts',(16.8055204004251,18.337646706947,-16.65478319563));
#92461=CARTESIAN_POINT('Ctrl Pts',(16.7997614702753,18.3505168054459,-16.6556288292752));
#92462=CARTESIAN_POINT('Ctrl Pts',(16.797902579604,18.3547075290473,-16.6559045945268));
#92463=CARTESIAN_POINT('Ctrl Pts',(16.7946195145981,18.3621742855265,-16.6563967248373));
#92464=CARTESIAN_POINT('Ctrl Pts',(16.7931900050555,18.3654479176277,-16.6566127596762));
#92465=CARTESIAN_POINT('Ctrl Pts',(16.7901344690081,18.3724937861814,-16.6570783321415));
#92466=CARTESIAN_POINT('Ctrl Pts',(16.7885111578161,18.3762670861491,-16.6573280244621));
#92467=CARTESIAN_POINT('Ctrl Pts',(16.7840607644922,18.3866952879818,-16.6580190455068));
#92468=CARTESIAN_POINT('Ctrl Pts',(16.7812568102554,18.3933599130058,-16.6584617404719));
#92469=CARTESIAN_POINT('Ctrl Pts',(16.7668566453678,18.4280837731999,-16.6607732919043));
#92470=CARTESIAN_POINT('Ctrl Pts',(16.7558316159281,18.4563740043379,-16.6626735625179));
#92471=CARTESIAN_POINT('Ctrl Pts',(16.7454194503294,18.4848895418246,-16.6645989754405));
#92472=CARTESIAN_POINT('Ctrl Pts',(16.7454194446555,18.4848895573635,-16.4437313838642));
#92473=CARTESIAN_POINT('Ctrl Pts',(16.7704615306514,18.4163074211586,-16.4397241110012));
#92474=CARTESIAN_POINT('Ctrl Pts',(16.7990388766678,18.349055408265,-16.4357751040702));
#92475=CARTESIAN_POINT('Ctrl Pts',(16.8846074405981,18.1735115759695,-16.4251562043927));
#92476=CARTESIAN_POINT('Ctrl Pts',(16.9475863594341,18.0684795667363,-16.4184725391856));
#92477=CARTESIAN_POINT('Ctrl Pts',(17.0262143222114,17.9598814560045,-16.4105598910851));
#92478=CARTESIAN_POINT('Ctrl Pts',(17.0332468354988,17.950338193115,-16.4098553651788));
#92479=CARTESIAN_POINT('Ctrl Pts',(17.0433668792879,17.936843892707,-16.4088452168993));
#92480=CARTESIAN_POINT('Ctrl Pts',(17.0463890177702,17.9328437865109,-16.4085440160231));
#92481=CARTESIAN_POINT('Ctrl Pts',(17.0516249495664,17.9259644438552,-16.4080228927674));
#92482=CARTESIAN_POINT('Ctrl Pts',(17.0538320188974,17.9230800700326,-16.4078034428587));
#92483=CARTESIAN_POINT('Ctrl Pts',(17.0581283780679,17.9174950850107,-16.4073766446614));
#92484=CARTESIAN_POINT('Ctrl Pts',(17.0602167830424,17.9147938433464,-16.4071693638787));
#92485=CARTESIAN_POINT('Ctrl Pts',(17.0658747510241,17.9075120340758,-16.4066083056037));
#92486=CARTESIAN_POINT('Ctrl Pts',(17.0694566109586,17.9029411222151,-16.4062536670681));
#92487=CARTESIAN_POINT('Ctrl Pts',(17.0828547584918,17.8859875158255,-16.4049293334138));
#92488=CARTESIAN_POINT('Ctrl Pts',(17.0927905037472,17.873700464655,-16.4039516191479));
#92489=CARTESIAN_POINT('Ctrl Pts',(17.1850072210732,17.7622361696263,-16.3949256851549));
#92490=CARTESIAN_POINT('Ctrl Pts',(17.2760386713513,17.6706630134185,-16.3863804075939));
#92491=CARTESIAN_POINT('Ctrl Pts',(17.4471373716444,17.5273815367175,-16.3716359364207));
#92492=CARTESIAN_POINT('Ctrl Pts',(17.5234275556216,17.4717175414131,-16.3654339514517));
#92493=CARTESIAN_POINT('Ctrl Pts',(17.6472805455279,17.3934601810411,-16.3560397924745));
#92494=CARTESIAN_POINT('Ctrl Pts',(17.6923971686405,17.3672336341904,-16.3527432610836));
#92495=CARTESIAN_POINT('Ctrl Pts',(17.7577913354779,17.3323870910632,-16.348142686415));
#92496=CARTESIAN_POINT('Ctrl Pts',(17.7773025027236,17.3223762223864,-16.3467915879511));
#92497=CARTESIAN_POINT('Ctrl Pts',(17.8120124089517,17.3052430828614,-16.3444252533818));
#92498=CARTESIAN_POINT('Ctrl Pts',(17.8271466380412,17.2979951514389,-16.3434057332562));
#92499=CARTESIAN_POINT('Ctrl Pts',(17.8497424354057,17.28750222027,-16.3419013132079));
#92500=CARTESIAN_POINT('Ctrl Pts',(17.8571388390056,17.2841191898847,-16.3414116549642));
#92501=CARTESIAN_POINT('Ctrl Pts',(17.8704014009748,17.2781452252445,-16.3405385643761));
#92502=CARTESIAN_POINT('Ctrl Pts',(17.876260150255,17.275538176017,-16.3401545813735));
#92503=CARTESIAN_POINT('Ctrl Pts',(17.8877713728649,17.2704784013072,-16.3394034363394));
#92504=CARTESIAN_POINT('Ctrl Pts',(17.8934228831066,17.2680236552739,-16.3390362081115));
#92505=CARTESIAN_POINT('Ctrl Pts',(17.9087987350939,17.2614247624792,-16.3380412601121));
#92506=CARTESIAN_POINT('Ctrl Pts',(17.9185436111592,17.2573286820976,-16.3374151805354));
#92507=CARTESIAN_POINT('Ctrl Pts',(17.9556042876434,17.2420765117757,-16.3350507499504));
#92508=CARTESIAN_POINT('Ctrl Pts',(17.9831223803184,17.2314186012617,-16.3333292111239));
#92509=CARTESIAN_POINT('Ctrl Pts',(18.0171056445599,17.2190673429564,-16.331241227544));
#92510=CARTESIAN_POINT('Ctrl Pts',(18.0233666816409,17.2168251041448,-16.3308581002547));
#92511=CARTESIAN_POINT('Ctrl Pts',(18.2107989234549,17.1506956085706,-16.3194341215848));
#92512=CARTESIAN_POINT('Ctrl Pts',(18.3998039003853,17.1117365839016,-16.3092858481144));
#92513=CARTESIAN_POINT('Ctrl Pts',(18.6540373129886,17.0945815900907,-16.2952817936928));
#92514=CARTESIAN_POINT('Ctrl Pts',(18.7167523310306,17.0931420523626,-16.2917894011348));
#92515=CARTESIAN_POINT('Ctrl Pts',(18.8103525060619,17.0951513036267,-16.2864042814848));
#92516=CARTESIAN_POINT('Ctrl Pts',(18.8412512065431,17.0964924065404,-16.2845982904104));
#92517=CARTESIAN_POINT('Ctrl Pts',(18.8792207313226,17.0989747272743,-16.2823321553682));
#92518=CARTESIAN_POINT('Ctrl Pts',(18.8863313914775,17.0994756792029,-16.2819057427643));
#92519=CARTESIAN_POINT('Ctrl Pts',(18.8975128599053,17.1003201963732,-16.2812318324158));
#92520=CARTESIAN_POINT('Ctrl Pts',(18.9015855106454,17.1006396552329,-16.2809856667422));
#92521=CARTESIAN_POINT('Ctrl Pts',(18.9092211361267,17.1012608361784,-16.2805227756422));
#92522=CARTESIAN_POINT('Ctrl Pts',(18.9127842797583,17.1015597978279,-16.2803062064237));
#92523=CARTESIAN_POINT('Ctrl Pts',(18.9209489220383,17.1022656782048,-16.2798086777473));
#92524=CARTESIAN_POINT('Ctrl Pts',(18.9255498444668,17.1026786308726,-16.2795273834362));
#92525=CARTESIAN_POINT('Ctrl Pts',(18.9398022677399,17.1040048854598,-16.2786532105473));
#92526=CARTESIAN_POINT('Ctrl Pts',(18.9494487144043,17.104969413954,-16.2780575664193));
#92527=CARTESIAN_POINT('Ctrl Pts',(19.0583922718588,17.1166187665741,-16.2712881671043));
#92528=CARTESIAN_POINT('Ctrl Pts',(19.1568094795274,17.1342500138841,-16.2647796484082));
#92529=CARTESIAN_POINT('Ctrl Pts',(19.4189277760569,17.200615039463,-16.2469646156926));
#92530=CARTESIAN_POINT('Ctrl Pts',(19.5786209928436,17.262306328343,-16.2356403865543));
#92531=CARTESIAN_POINT('Ctrl Pts',(19.7551327423921,17.3563192144771,-16.2231066089301));
#92532=CARTESIAN_POINT('Ctrl Pts',(19.780785029331,17.370675536726,-16.2212824452972));
#92533=CARTESIAN_POINT('Ctrl Pts',(19.8245078514859,17.3963551793112,-16.2181680336639));
#92534=CARTESIAN_POINT('Ctrl Pts',(19.842721106416,17.4074255602496,-16.2168690578628));
#92535=CARTESIAN_POINT('Ctrl Pts',(19.8683808270902,17.4235576727887,-16.215036066827));
#92536=CARTESIAN_POINT('Ctrl Pts',(19.8759665198765,17.4283944896968,-16.2144938126804));
#92537=CARTESIAN_POINT('Ctrl Pts',(19.8889995923516,17.4368220205085,-16.2135614369659));
#92538=CARTESIAN_POINT('Ctrl Pts',(19.8944615848521,17.4403898021285,-16.213170469153));
#92539=CARTESIAN_POINT('Ctrl Pts',(19.9048879955412,17.447269319616,-16.2124236884958));
#92540=CARTESIAN_POINT('Ctrl Pts',(19.9098550657846,17.4505769041444,-16.2120677251431));
#92541=CARTESIAN_POINT('Ctrl Pts',(19.922734539108,17.4592322078263,-16.2111441531797));
#92542=CARTESIAN_POINT('Ctrl Pts',(19.930624916454,17.464612581347,-16.2105777819303));
#92543=CARTESIAN_POINT('Ctrl Pts',(19.9574051396603,17.4831404764714,-16.2086533239791));
#92544=CARTESIAN_POINT('Ctrl Pts',(19.9761172950283,17.4965428394698,-16.207304948819));
#92545=CARTESIAN_POINT('Ctrl Pts',(20.1353166627209,17.6145423851928,-16.1957903035545));
#92546=CARTESIAN_POINT('Ctrl Pts',(20.2625385652158,17.7358925886438,-16.1863715732034));
#92547=CARTESIAN_POINT('Ctrl Pts',(20.4285658908881,17.9390935895098,-16.1720947011483));
#92548=CARTESIAN_POINT('Ctrl Pts',(20.4795301237799,18.0099914014938,-16.1673195255445));
#92549=CARTESIAN_POINT('Ctrl Pts',(20.5461419212577,18.1158900825681,-16.1601770607969));
#92550=CARTESIAN_POINT('Ctrl Pts',(20.5654462905767,18.1484896904844,-16.1579766778086));
#92551=CARTESIAN_POINT('Ctrl Pts',(20.5875478672095,18.1882064304733,-16.1552724158058));
#92552=CARTESIAN_POINT('Ctrl Pts',(20.591195711937,18.1948452551236,-16.154819614514));
#92553=CARTESIAN_POINT('Ctrl Pts',(20.5968024601485,18.2051801891155,-16.154113300508));
#92554=CARTESIAN_POINT('Ctrl Pts',(20.5987862129881,18.208862845386,-16.1538613409515));
#92555=CARTESIAN_POINT('Ctrl Pts',(20.6024397918604,18.2156937936839,-16.1533934227245));
#92556=CARTESIAN_POINT('Ctrl Pts',(20.6041125877399,18.2188404318184,-16.1531776561949));
#92557=CARTESIAN_POINT('Ctrl Pts',(20.6078699860158,18.2259516060288,-16.1526895418979));
#92558=CARTESIAN_POINT('Ctrl Pts',(20.6099499438573,18.2299185200787,-16.1524169074041));
#92559=CARTESIAN_POINT('Ctrl Pts',(20.6160334232944,18.2416110648502,-16.1516123703569));
#92560=CARTESIAN_POINT('Ctrl Pts',(20.6200018641408,18.2493547033928,-16.1510783419754));
#92561=CARTESIAN_POINT('Ctrl Pts',(20.647809630442,18.3044503692619,-16.1472713998582));
#92562=CARTESIAN_POINT('Ctrl Pts',(20.6699085752681,18.3526547876637,-16.1439026066277));
#92563=CARTESIAN_POINT('Ctrl Pts',(20.6974105989166,18.419124903479,-16.1392545425674));
#92564=CARTESIAN_POINT('Ctrl Pts',(20.7044128210968,18.4367128227123,-16.1380243728112));
#92565=CARTESIAN_POINT('Ctrl Pts',(20.7281825343384,18.498828144907,-16.1336838334092));
#92566=CARTESIAN_POINT('Ctrl Pts',(20.7436837153178,18.5438239556507,-16.130547154643));
#92567=CARTESIAN_POINT('Ctrl Pts',(20.7897747142654,18.6938523942022,-16.1201795341099));
#92568=CARTESIAN_POINT('Ctrl Pts',(20.8137460009862,18.8007423255791,-16.1129474872608));
#92569=CARTESIAN_POINT('Ctrl Pts',(20.8372085215249,18.9635374632004,-16.1023754190192));
#92570=CARTESIAN_POINT('Ctrl Pts',(20.8429361007121,19.018352301346,-16.0988870151962));
#92571=CARTESIAN_POINT('Ctrl Pts',(20.8487493996785,19.1075575720974,-16.0933304765121));
#92572=CARTESIAN_POINT('Ctrl Pts',(20.8501478196467,19.1418336717667,-16.091223920679));
#92573=CARTESIAN_POINT('Ctrl Pts',(20.8508908250243,19.1869366535892,-16.0884877295449));
#92574=CARTESIAN_POINT('Ctrl Pts',(20.8509860900701,19.1977443994115,-16.0878347601204));
#92575=CARTESIAN_POINT('Ctrl Pts',(20.8510065598351,19.2154504384766,-16.0867693029909));
#92576=CARTESIAN_POINT('Ctrl Pts',(20.850980821094,19.2223483769558,-16.086355286078));
#92577=CARTESIAN_POINT('Ctrl Pts',(20.850865717936,19.2357026787889,-16.0855557757483));
#92578=CARTESIAN_POINT('Ctrl Pts',(20.8507805291747,19.2421589929963,-16.0851701560413));
#92579=CARTESIAN_POINT('Ctrl Pts',(20.8505155754932,19.2570684786624,-16.0842817148123));
#92580=CARTESIAN_POINT('Ctrl Pts',(20.850314704346,19.2655212010512,-16.0837795594562));
#92581=CARTESIAN_POINT('Ctrl Pts',(20.8496380997534,19.2882570949629,-16.0824328698369));
#92582=CARTESIAN_POINT('Ctrl Pts',(20.8490683645714,19.3025371834458,-16.0815912775324));
#92583=CARTESIAN_POINT('Ctrl Pts',(20.8425104361114,19.4335805095935,-16.0739047273808));
#92584=CARTESIAN_POINT('Ctrl Pts',(20.8270036818209,19.5496727052252,-16.0673769189932));
#92585=CARTESIAN_POINT('Ctrl Pts',(20.7671076590146,19.8231615861361,-16.0520504590556));
#92586=CARTESIAN_POINT('Ctrl Pts',(20.7139537705473,19.977837431565,-16.0434357244137));
#92587=CARTESIAN_POINT('Ctrl Pts',(20.6297053860372,20.1538811836281,-16.0322254754236));
#92588=CARTESIAN_POINT('Ctrl Pts',(20.6151600109521,20.1825763462623,-16.0303487372091));
#92589=CARTESIAN_POINT('Ctrl Pts',(20.5965589974672,20.2172877598065,-16.0280038204065));
#92590=CARTESIAN_POINT('Ctrl Pts',(20.5931180759991,20.2236307573174,-16.0275722127252));
#92591=CARTESIAN_POINT('Ctrl Pts',(20.5876692368418,20.2335537676982,-16.0268919176751));
#92592=CARTESIAN_POINT('Ctrl Pts',(20.5856831850314,20.2371458127681,-16.0266446047377));
#92593=CARTESIAN_POINT('Ctrl Pts',(20.5819489223078,20.2438535930472,-16.0261807592261));
#92594=CARTESIAN_POINT('Ctrl Pts',(20.5802032662988,20.2469706863496,-16.0259643901107));
#92595=CARTESIAN_POINT('Ctrl Pts',(20.5761971777473,20.2540817896673,-16.0254689128982));
#92596=CARTESIAN_POINT('Ctrl Pts',(20.5739316503172,20.2580728641697,-16.0251894802629));
#92597=CARTESIAN_POINT('Ctrl Pts',(20.5679813929563,20.2684762149334,-16.0244576327782));
#92598=CARTESIAN_POINT('Ctrl Pts',(20.5642760439421,20.2748765408433,-16.0240039368438));
#92599=CARTESIAN_POINT('Ctrl Pts',(20.5397023474197,20.3168148457175,-16.0210090073442));
#92600=CARTESIAN_POINT('Ctrl Pts',(20.5178350509524,20.3517538891273,-16.0184094103354));
#92601=CARTESIAN_POINT('Ctrl Pts',(20.4893125920036,20.3944992071165,-16.01511743289));
#92602=CARTESIAN_POINT('Ctrl Pts',(20.483600294008,20.4029276295792,-16.014462753299));
#92603=CARTESIAN_POINT('Ctrl Pts',(20.4774536526555,20.4118575251865,-16.0137634109665));
#92604=CARTESIAN_POINT('Ctrl Pts',(20.4770795501952,20.4124004812903,-16.0137208668999));
#92605=CARTESIAN_POINT('Ctrl Pts',(20.4637375587464,20.431745119707,-16.0122042876288));
#92606=CARTESIAN_POINT('Ctrl Pts',(20.4504668125158,20.4503354261383,-16.0107197946073));
#92607=CARTESIAN_POINT('Ctrl Pts',(20.4097658760076,20.5054433002699,-16.0062448422303));
#92608=CARTESIAN_POINT('Ctrl Pts',(20.3814524633525,20.5412912911306,-16.0032337198904));
#92609=CARTESIAN_POINT('Ctrl Pts',(20.2814844904335,20.6597714222965,-15.9929934764379));
#92610=CARTESIAN_POINT('Ctrl Pts',(20.2045911633877,20.7377652009908,-15.985762897092));
#92611=CARTESIAN_POINT('Ctrl Pts',(20.0804339735937,20.8455753752534,-15.9751939111193));
#92612=CARTESIAN_POINT('Ctrl Pts',(20.0374614049651,20.8800447231658,-15.9717071118169));
#92613=CARTESIAN_POINT('Ctrl Pts',(19.9656280011274,20.9331954211171,-15.9661528296056));
#92614=CARTESIAN_POINT('Ctrl Pts',(19.9375729784018,20.952917593733,-15.9640469646169));
#92615=CARTESIAN_POINT('Ctrl Pts',(19.9000608371231,20.9779487560198,-15.9613115259344));
#92616=CARTESIAN_POINT('Ctrl Pts',(19.8910258432682,20.9838781647546,-15.9606586341646));
#92617=CARTESIAN_POINT('Ctrl Pts',(19.8761502290105,20.9934784518513,-15.9595932712653));
#92618=CARTESIAN_POINT('Ctrl Pts',(19.8703364510601,20.9971903730249,-15.9591792714499));
#92619=CARTESIAN_POINT('Ctrl Pts',(19.8590454231376,21.0043219140586,-15.9583797716986));
#92620=CARTESIAN_POINT('Ctrl Pts',(19.8535704726723,21.0077450152183,-15.9579941455898));
#92621=CARTESIAN_POINT('Ctrl Pts',(19.8408898479131,21.0155928522036,-15.957105657542));
#92622=CARTESIAN_POINT('Ctrl Pts',(19.8336731230668,21.0199995918204,-15.9566034619942));
#92623=CARTESIAN_POINT('Ctrl Pts',(19.8141869538748,21.0317387072876,-15.9552565934069));
#92624=CARTESIAN_POINT('Ctrl Pts',(19.8018692003457,21.0389903395289,-15.9544148635639));
#92625=CARTESIAN_POINT('Ctrl Pts',(19.687971681656,21.1044991982377,-15.9467174738565));
#92626=CARTESIAN_POINT('Ctrl Pts',(19.5817897004939,21.1543628316632,-15.9401800358359));
#92627=CARTESIAN_POINT('Ctrl Pts',(19.3186486453608,21.2522374761913,-15.9248116575232));
#92628=CARTESIAN_POINT('Ctrl Pts',(19.1592046940596,21.2913012269958,-15.9161664072812));
#92629=CARTESIAN_POINT('Ctrl Pts',(18.9656472654506,21.3155234756884,-15.9049530471375));
#92630=CARTESIAN_POINT('Ctrl Pts',(18.9343369906131,21.3187344156688,-15.9031159327262));
#92631=CARTESIAN_POINT('Ctrl Pts',(18.8958240931573,21.3218181674089,-15.9008151267591));
#92632=CARTESIAN_POINT('Ctrl Pts',(18.8886767214384,21.3223539451003,-15.900386401206));
#92633=CARTESIAN_POINT('Ctrl Pts',(18.8774430127991,21.32313869371,-15.8997096479797));
#92634=CARTESIAN_POINT('Ctrl Pts',(18.8733583629199,21.3234121296327,-15.8994629711669));
#92635=CARTESIAN_POINT('Ctrl Pts',(18.8657059533733,21.3239021079378,-15.898999657603));
#92636=CARTESIAN_POINT('Ctrl Pts',(18.8621384297138,21.3241214631538,-15.8987831802999));
#92637=CARTESIAN_POINT('Ctrl Pts',(18.8539725030067,21.324602803852,-15.8982865782145));
#92638=CARTESIAN_POINT('Ctrl Pts',(18.8493738034868,21.3248588170622,-15.8980061232282));
#92639=CARTESIAN_POINT('Ctrl Pts',(18.8351628067134,21.3256034432128,-15.8971370918124));
#92640=CARTESIAN_POINT('Ctrl Pts',(18.8255481419381,21.3260415043647,-15.8965457955876));
#92641=CARTESIAN_POINT('Ctrl Pts',(18.7294004275695,21.3297653531511,-15.8906016342087));
#92642=CARTESIAN_POINT('Ctrl Pts',(18.6427551834193,21.3278038852054,-15.8849957737045));
#92643=CARTESIAN_POINT('Ctrl Pts',(18.4300104794483,21.3099017019319,-15.8709781227803));
#92644=CARTESIAN_POINT('Ctrl Pts',(18.304739685429,21.287905664406,-15.8625167854829));
#92645=CARTESIAN_POINT('Ctrl Pts',(18.0889889683362,21.2296554581317,-15.8480526034237));
#92646=CARTESIAN_POINT('Ctrl Pts',(17.9976063531014,21.1981431813898,-15.8419579312411));
#92647=CARTESIAN_POINT('Ctrl Pts',(17.8952172026777,21.1547968602301,-15.8351790078744));
#92648=CARTESIAN_POINT('Ctrl Pts',(17.8818109215526,21.148956812298,-15.8342922488543));
#92649=CARTESIAN_POINT('Ctrl Pts',(17.8614116482803,21.1398178554646,-15.832943980679));
#92650=CARTESIAN_POINT('Ctrl Pts',(17.8543746314943,21.1366188523872,-15.8324790671705));
#92651=CARTESIAN_POINT('Ctrl Pts',(17.8415803413249,21.1307178428823,-15.8316340838682));
#92652=CARTESIAN_POINT('Ctrl Pts',(17.8358174453569,21.1280283105296,-15.8312535902115));
#92653=CARTESIAN_POINT('Ctrl Pts',(17.8233758133189,21.1221534058359,-15.8304323332899));
#92654=CARTESIAN_POINT('Ctrl Pts',(17.8167014656391,21.1189588965691,-15.8299918922878));
#92655=CARTESIAN_POINT('Ctrl Pts',(17.7985847175492,21.1101707301395,-15.8287966188649));
#92656=CARTESIAN_POINT('Ctrl Pts',(17.7871757109797,21.1045086451464,-15.8280441741482));
#92657=CARTESIAN_POINT('Ctrl Pts',(17.7311353452366,21.0760636563785,-15.8243486701561));
#92658=CARTESIAN_POINT('Ctrl Pts',(17.6872694614211,21.051803009335,-15.8214579772666));
#92659=CARTESIAN_POINT('Ctrl Pts',(17.4954797346555,20.9366559798244,-15.8087586078297));
#92660=CARTESIAN_POINT('Ctrl Pts',(17.3582177129612,20.8293460645849,-15.7995651219046));
#92661=CARTESIAN_POINT('Ctrl Pts',(17.19129710037,20.6620992066969,-15.786578876898));
#92662=CARTESIAN_POINT('Ctrl Pts',(17.1489969925824,20.615772387948,-15.7830863884505));
#92663=CARTESIAN_POINT('Ctrl Pts',(17.0889996927197,20.5438988842907,-15.7777011350884));
#92664=CARTESIAN_POINT('Ctrl Pts',(17.0697048264685,20.5197271659977,-15.7758951112547));
#92665=CARTESIAN_POINT('Ctrl Pts',(17.0466234949472,20.4894757894566,-15.773628939708));
#92666=CARTESIAN_POINT('Ctrl Pts',(17.0423282298531,20.4837868764361,-15.7732025246463));
#92667=CARTESIAN_POINT('Ctrl Pts',(17.0356167548365,20.4748037986237,-15.7725286112769));
#92668=CARTESIAN_POINT('Ctrl Pts',(17.0331811635899,20.4715240870096,-15.7722824450599));
#92669=CARTESIAN_POINT('Ctrl Pts',(17.0286315565118,20.4653604975651,-15.7718195535131));
#92670=CARTESIAN_POINT('Ctrl Pts',(17.0265153489592,20.4624783065149,-15.7716029843948));
#92671=CARTESIAN_POINT('Ctrl Pts',(17.0216819502108,20.4558603277475,-15.7711054567143));
#92672=CARTESIAN_POINT('Ctrl Pts',(17.0189696857099,20.4521210091549,-15.7708241633042));
#92673=CARTESIAN_POINT('Ctrl Pts',(17.0106032987982,20.4405067282988,-15.769949995944));
#92674=CARTESIAN_POINT('Ctrl Pts',(17.0049911091582,20.432601912176,-15.7693543564931));
#92675=CARTESIAN_POINT('Ctrl Pts',(16.942141667551,20.3427772303528,-15.762580978144));
#92676=CARTESIAN_POINT('Ctrl Pts',(16.8907261578416,20.2569506599535,-15.7560680511294));
#92677=CARTESIAN_POINT('Ctrl Pts',(16.768406338946,20.0155354424814,-15.738236566643));
#92678=CARTESIAN_POINT('Ctrl Pts',(16.7099350762936,19.8544398915282,-15.7269007125148));
#92679=CARTESIAN_POINT('Ctrl Pts',(16.6614520672809,19.6448237544999,-15.7134187937563));
#92680=CARTESIAN_POINT('Ctrl Pts',(16.6528139418684,19.6012858439423,-15.7106795639875));
#92681=CARTESIAN_POINT('Ctrl Pts',(16.6436144406144,19.5458388846826,-15.7072652732538));
#92682=CARTESIAN_POINT('Ctrl Pts',(16.6417764781134,19.5341557038691,-15.706549965101));
#92683=CARTESIAN_POINT('Ctrl Pts',(16.6389885125918,19.51541190343,-15.7054088058363));
#92684=CARTESIAN_POINT('Ctrl Pts',(16.6379760960099,19.5083609509589,-15.7049809854188));
#92685=CARTESIAN_POINT('Ctrl Pts',(16.6361227657874,19.4949735293922,-15.7041714108607));
#92686=CARTESIAN_POINT('Ctrl Pts',(16.635274926426,19.4886381136652,-15.7037894418225));
#92687=CARTESIAN_POINT('Ctrl Pts',(16.6334140698746,19.4742372053294,-15.702923765898));
#92688=CARTESIAN_POINT('Ctrl Pts',(16.6324187836035,19.4661694923306,-15.7024406236861));
#92689=CARTESIAN_POINT('Ctrl Pts',(16.6299653959363,19.4452937279088,-15.701195073411));
#92690=CARTESIAN_POINT('Ctrl Pts',(16.6285777518862,19.4324776155075,-15.7004348865106));
#92691=CARTESIAN_POINT('Ctrl Pts',(16.6203967177256,19.3498752954838,-15.6955629102487));
#92692=CARTESIAN_POINT('Ctrl Pts',(16.616956381725,19.2797966609927,-15.691558250133));
#92693=CARTESIAN_POINT('Ctrl Pts',(16.6171212268841,19.0172834136081,-15.676859263182));
#92694=CARTESIAN_POINT('Ctrl Pts',(16.6434647892515,18.8258343582239,-15.6668249337217));
#92695=CARTESIAN_POINT('Ctrl Pts',(16.7087052425926,18.5926572672549,-15.6531662107904));
#92696=CARTESIAN_POINT('Ctrl Pts',(16.723802096131,18.5452146498781,-15.6503027130819));
#92697=CARTESIAN_POINT('Ctrl Pts',(16.742161444939,18.4938591918365,-15.6470652126431));
#92698=CARTESIAN_POINT('Ctrl Pts',(16.7437828789803,18.489371578843,-15.6467811375154));
#92699=CARTESIAN_POINT('Ctrl Pts',(16.7454194503191,18.4848895418528,-15.6464962064494));
#92700=CARTESIAN_POINT('Origin',(18.734,19.211,0.));
#92701=CARTESIAN_POINT('',(16.7454194448477,18.4848895568371,-14.8438385225655));
#92702=CARTESIAN_POINT('',(16.7486736478041,18.4860706551708,-15.066381399058));
#92703=CARTESIAN_POINT('',(16.7454194503191,18.4848895418526,0.));
#92704=CARTESIAN_POINT('',(16.6156459487826,19.212740575031,-15.1109429532718));
#92705=CARTESIAN_POINT('Ctrl Pts',(16.7486736478041,18.4860706551708,-15.066381399058));
#92706=CARTESIAN_POINT('Ctrl Pts',(16.6638907080669,18.7190472863516,-15.0812352504626));
#92707=CARTESIAN_POINT('Ctrl Pts',(16.6178442115102,18.9662441554235,-15.0960891018672));
#92708=CARTESIAN_POINT('Ctrl Pts',(16.6156459487826,19.212740575031,-15.1109429532718));
#92709=CARTESIAN_POINT('Ctrl Pts',(16.6170007608289,19.212794811659,-15.1101643053096));
#92710=CARTESIAN_POINT('Ctrl Pts',(16.6170691197604,19.2934248907551,-15.1145731285289));
#92711=CARTESIAN_POINT('Ctrl Pts',(16.6217438740534,19.3739800238093,-15.1190366797522));
#92712=CARTESIAN_POINT('Ctrl Pts',(16.6337248047666,19.4776387155272,-15.1250697176005));
#92713=CARTESIAN_POINT('Ctrl Pts',(16.6368453917013,19.5011629633464,-15.1264584526702));
#92714=CARTESIAN_POINT('Ctrl Pts',(16.6412432748791,19.5305211890863,-15.1282216951713));
#92715=CARTESIAN_POINT('Ctrl Pts',(16.6421508377164,19.5364098664599,-15.1285768878127));
#92716=CARTESIAN_POINT('Ctrl Pts',(16.643715780129,19.5462867698596,-15.1291753145913));
#92717=CARTESIAN_POINT('Ctrl Pts',(16.6443597513821,19.5502771265929,-15.1294178177132));
#92718=CARTESIAN_POINT('Ctrl Pts',(16.6455594680068,19.5575781495653,-15.1298629008675));
#92719=CARTESIAN_POINT('Ctrl Pts',(16.6461116697319,19.5608893959485,-15.1300652817493));
#92720=CARTESIAN_POINT('Ctrl Pts',(16.6472681665132,19.567724031502,-15.130484112733));
#92721=CARTESIAN_POINT('Ctrl Pts',(16.6478735058963,19.5712471782848,-15.1307006235895));
#92722=CARTESIAN_POINT('Ctrl Pts',(16.64928005852,19.5793110447164,-15.1311975665018));
#92723=CARTESIAN_POINT('Ctrl Pts',(16.6500871823861,19.5838506775108,-15.1314783304732));
#92724=CARTESIAN_POINT('Ctrl Pts',(16.6526294587065,19.5978834459161,-15.1323492524446));
#92725=CARTESIAN_POINT('Ctrl Pts',(16.6544146697914,19.6073672251524,-15.1329421470191));
#92726=CARTESIAN_POINT('Ctrl Pts',(16.673431573657,19.7047264393825,-15.139070638307));
#92727=CARTESIAN_POINT('Ctrl Pts',(16.6961558788501,19.7914271088415,-15.1448764765017));
#92728=CARTESIAN_POINT('Ctrl Pts',(16.738599780215,19.9196167563596,-15.1537504328869));
#92729=CARTESIAN_POINT('Ctrl Pts',(16.7542920844716,19.9623429485463,-15.1567594503444));
#92730=CARTESIAN_POINT('Ctrl Pts',(16.7857100315866,20.0400495149138,-15.1622978990167));
#92731=CARTESIAN_POINT('Ctrl Pts',(16.8010330167755,20.0751733743205,-15.1648270609592));
#92732=CARTESIAN_POINT('Ctrl Pts',(16.8576523026906,20.1959061170435,-15.1735859373226));
#92733=CARTESIAN_POINT('Ctrl Pts',(16.9037553976654,20.279142813405,-15.1797350589487));
#92734=CARTESIAN_POINT('Ctrl Pts',(16.98037113813,20.3978496151008,-15.1886008559529));
#92735=CARTESIAN_POINT('Ctrl Pts',(17.0067076175732,20.4358623371365,-15.1914572270433));
#92736=CARTESIAN_POINT('Ctrl Pts',(17.0414157633168,20.4826097334158,-15.194994936695));
#92737=CARTESIAN_POINT('Ctrl Pts',(17.0486437876414,20.4921741330187,-15.1957201364725));
#92738=CARTESIAN_POINT('Ctrl Pts',(17.0603173995666,20.5073513426466,-15.1968733046793));
#92739=CARTESIAN_POINT('Ctrl Pts',(17.0647108123106,20.51300378663,-15.1973033161713));
#92740=CARTESIAN_POINT('Ctrl Pts',(17.0730769268785,20.5236554448443,-15.1981147104128));
#92741=CARTESIAN_POINT('Ctrl Pts',(17.0770437298117,20.5286591713228,-15.198496321254));
#92742=CARTESIAN_POINT('Ctrl Pts',(17.0860738393375,20.5399444917881,-15.1993580650651));
#92743=CARTESIAN_POINT('Ctrl Pts',(17.0911505572635,20.5462152652305,-15.1998376533312));
#92744=CARTESIAN_POINT('Ctrl Pts',(17.1062386171615,20.5646357397032,-15.2012488100003));
#92745=CARTESIAN_POINT('Ctrl Pts',(17.1163499124345,20.5767031337094,-15.2021763243838));
#92746=CARTESIAN_POINT('Ctrl Pts',(17.2076552505965,20.6832352123291,-15.2103952542774));
#92747=CARTESIAN_POINT('Ctrl Pts',(17.2969087698296,20.7704805616849,-15.2173237787246));
#92748=CARTESIAN_POINT('Ctrl Pts',(17.5230057614327,20.9554937227271,-15.2332793356579));
#92749=CARTESIAN_POINT('Ctrl Pts',(17.6648036943985,21.0458212970044,-15.2421392555806));
#92750=CARTESIAN_POINT('Ctrl Pts',(17.8351453836605,21.1278237449123,-15.2531373168278));
#92751=CARTESIAN_POINT('Ctrl Pts',(17.8546924769311,21.1368689179489,-15.2544048484744));
#92752=CARTESIAN_POINT('Ctrl Pts',(17.8801232774212,21.1481688446537,-15.2560652200103));
#92753=CARTESIAN_POINT('Ctrl Pts',(17.8858845389524,21.1506981086003,-15.2564421137673));
#92754=CARTESIAN_POINT('Ctrl Pts',(17.8947422388003,21.1545397397834,-15.257022836009));
#92755=CARTESIAN_POINT('Ctrl Pts',(17.8978307301784,21.1558704999805,-15.2572255563272));
#92756=CARTESIAN_POINT('Ctrl Pts',(17.9042045086151,21.1585988264718,-15.2576444238103));
#92757=CARTESIAN_POINT('Ctrl Pts',(17.9074901355794,21.1599954309256,-15.2578606286241));
#92758=CARTESIAN_POINT('Ctrl Pts',(17.9149829265378,21.1631579987719,-15.2583543127009));
#92759=CARTESIAN_POINT('Ctrl Pts',(17.9191922603767,21.1649186690701,-15.2586321074155));
#92760=CARTESIAN_POINT('Ctrl Pts',(17.9301580868714,21.1694638323502,-15.2593569044156));
#92761=CARTESIAN_POINT('Ctrl Pts',(17.9369232980745,21.1722269454673,-15.2598051486424));
#92762=CARTESIAN_POINT('Ctrl Pts',(17.9802281062826,21.1896528437242,-15.2626807311095));
#92763=CARTESIAN_POINT('Ctrl Pts',(18.017153974243,21.2033279007886,-15.2651613189248));
#92764=CARTESIAN_POINT('Ctrl Pts',(18.2352196800195,21.2772391545958,-15.279889625781));
#92765=CARTESIAN_POINT('Ctrl Pts',(18.4234627722836,21.3137848053859,-15.292819965755));
#92766=CARTESIAN_POINT('Ctrl Pts',(18.6690771857391,21.3277214028344,-15.3086327479154));
#92767=CARTESIAN_POINT('Ctrl Pts',(18.7241880123992,21.3286942684755,-15.3121215554525));
#92768=CARTESIAN_POINT('Ctrl Pts',(18.8135709767503,21.3267821271883,-15.3176786619517));
#92769=CARTESIAN_POINT('Ctrl Pts',(18.8478425684395,21.3252151347389,-15.3197853916697));
#92770=CARTESIAN_POINT('Ctrl Pts',(18.8928443013813,21.3220599954916,-15.3225217722703));
#92771=CARTESIAN_POINT('Ctrl Pts',(18.903620215058,21.3212215064005,-15.3231747613143));
#92772=CARTESIAN_POINT('Ctrl Pts',(18.921262260065,21.3197127418703,-15.3242402423033));
#92773=CARTESIAN_POINT('Ctrl Pts',(18.9281322748977,21.3190913745296,-15.3246542635876));
#92774=CARTESIAN_POINT('Ctrl Pts',(18.941426786433,21.3178233950745,-15.3254537767271));
#92775=CARTESIAN_POINT('Ctrl Pts',(18.94785159488,21.3171809481989,-15.3258393949022));
#92776=CARTESIAN_POINT('Ctrl Pts',(18.9626822979287,21.3156293948725,-15.3267278245541));
#92777=CARTESIAN_POINT('Ctrl Pts',(18.971085922556,21.31469930162,-15.3272299699215));
#92778=CARTESIAN_POINT('Ctrl Pts',(18.9936776825545,21.3120618058809,-15.3285766148951));
#92779=CARTESIAN_POINT('Ctrl Pts',(19.0078546294512,21.3102610289786,-15.3294181728522));
#92780=CARTESIAN_POINT('Ctrl Pts',(19.1377965712587,21.2924168454141,-15.337102041364));
#92781=CARTESIAN_POINT('Ctrl Pts',(19.2520722511782,21.2669557788185,-15.3436274674306));
#92782=CARTESIAN_POINT('Ctrl Pts',(19.5191932517011,21.1837376537684,-15.3589439081253));
#92783=CARTESIAN_POINT('Ctrl Pts',(19.6685807115964,21.1175070858719,-15.3675514160382));
#92784=CARTESIAN_POINT('Ctrl Pts',(19.8367388909741,21.0184018770823,-15.3787610362288));
#92785=CARTESIAN_POINT('Ctrl Pts',(19.8642150773718,21.0013486332106,-15.3806472681951));
#92786=CARTESIAN_POINT('Ctrl Pts',(19.8973404289251,20.9797227842018,-15.3830027492314));
#92787=CARTESIAN_POINT('Ctrl Pts',(19.9033722574255,20.9757407064675,-15.3834350373594));
#92788=CARTESIAN_POINT('Ctrl Pts',(19.9127993871593,20.9694475747342,-15.3841161685256));
#92789=CARTESIAN_POINT('Ctrl Pts',(19.916208621062,20.9671573516867,-15.3843636315422));
#92790=CARTESIAN_POINT('Ctrl Pts',(19.9225706730188,20.9628565913669,-15.3848276035793));
#92791=CARTESIAN_POINT('Ctrl Pts',(19.9255250739641,20.960848495994,-15.3850439481982));
#92792=CARTESIAN_POINT('Ctrl Pts',(19.9322601965055,20.9562456926736,-15.3855391646632));
#92793=CARTESIAN_POINT('Ctrl Pts',(19.9360375663805,20.9536461816506,-15.38581835973));
#92794=CARTESIAN_POINT('Ctrl Pts',(19.9476314937909,20.9456118395016,-15.3866797057842));
#92795=CARTESIAN_POINT('Ctrl Pts',(19.9554197332402,20.940136623848,-15.3872645088872));
#92796=CARTESIAN_POINT('Ctrl Pts',(20.0608327242514,20.8649626507338,-15.3952614107075));
#92797=CARTESIAN_POINT('Ctrl Pts',(20.1523877659229,20.7871494252094,-15.4031531095498));
#92798=CARTESIAN_POINT('Ctrl Pts',(20.3135179904146,20.6247401417072,-15.4182672139133));
#92799=CARTESIAN_POINT('Ctrl Pts',(20.3841163943823,20.5416606007797,-15.4254618019288));
#92800=CARTESIAN_POINT('Ctrl Pts',(20.4919507452078,20.3929060549428,-15.4372653250561));
#92801=CARTESIAN_POINT('Ctrl Pts',(20.5326447102117,20.3300049524239,-15.4419746596193));
#92802=CARTESIAN_POINT('Ctrl Pts',(20.5792769856146,20.2487835409625,-15.4477119319991));
#92803=CARTESIAN_POINT('Ctrl Pts',(20.5884126207073,20.2323695214722,-15.4488547983053));
#92804=CARTESIAN_POINT('Ctrl Pts',(20.6013870623139,20.208310213105,-15.4505064814297));
#92805=CARTESIAN_POINT('Ctrl Pts',(20.6053997217216,20.2007601661773,-15.4510214756272));
#92806=CARTESIAN_POINT('Ctrl Pts',(20.6123583853641,20.1874734301005,-15.4519220347232));
#92807=CARTESIAN_POINT('Ctrl Pts',(20.6153241017789,20.1817472426193,-15.4523082940495));
#92808=CARTESIAN_POINT('Ctrl Pts',(20.6210346052342,20.1705969733215,-15.4530568754688));
#92809=CARTESIAN_POINT('Ctrl Pts',(20.623782281851,20.165174449955,-15.453419296536));
#92810=CARTESIAN_POINT('Ctrl Pts',(20.6302989861685,20.1521752043832,-15.4542842819653));
#92811=CARTESIAN_POINT('Ctrl Pts',(20.6340460340923,20.1445875330033,-15.4547860742798));
#92812=CARTESIAN_POINT('Ctrl Pts',(20.6474264613079,20.1170782740257,-15.4565943426743));
#92813=CARTESIAN_POINT('Ctrl Pts',(20.6567930564118,20.0970279782003,-15.4578915650937));
#92814=CARTESIAN_POINT('Ctrl Pts',(20.7416650400087,19.9076620830962,-15.4699604304115));
#92815=CARTESIAN_POINT('Ctrl Pts',(20.7949366097104,19.7292695186358,-15.4798776729096));
#92816=CARTESIAN_POINT('Ctrl Pts',(20.8370036304495,19.466946153904,-15.4943601181923));
#92817=CARTESIAN_POINT('Ctrl Pts',(20.8451946785674,19.3870332888556,-15.4987741917299));
#92818=CARTESIAN_POINT('Ctrl Pts',(20.850461770287,19.2708271156551,-15.5054278730004));
#92819=CARTESIAN_POINT('Ctrl Pts',(20.8511737220716,19.2347653081696,-15.5075256032415));
#92820=CARTESIAN_POINT('Ctrl Pts',(20.8509209260533,19.1912371681383,-15.5101160388122));
#92821=CARTESIAN_POINT('Ctrl Pts',(20.8508380342263,19.1837693230324,-15.5105625389141));
#92822=CARTESIAN_POINT('Ctrl Pts',(20.8506474517536,19.1721429693674,-15.5112611222685));
#92823=CARTESIAN_POINT('Ctrl Pts',(20.85056701431,19.1679839902409,-15.5115117064976));
#92824=CARTESIAN_POINT('Ctrl Pts',(20.8503948597539,19.1602603412614,-15.5119783873891));
#92825=CARTESIAN_POINT('Ctrl Pts',(20.8503063939365,19.1566956563464,-15.512194300298));
#92826=CARTESIAN_POINT('Ctrl Pts',(20.8500856425717,19.1486229796412,-15.512684448632));
#92827=CARTESIAN_POINT('Ctrl Pts',(20.8499479582416,19.144115199711,-15.512958981371));
#92828=CARTESIAN_POINT('Ctrl Pts',(20.849497605133,19.1307684033944,-15.5137742286541));
#92829=CARTESIAN_POINT('Ctrl Pts',(20.8491439508148,19.1219309959322,-15.5143171527537));
#92830=CARTESIAN_POINT('Ctrl Pts',(20.8461180363622,19.0565708177643,-15.5183543269264));
#92831=CARTESIAN_POINT('Ctrl Pts',(20.8412360822994,19.0001781445165,-15.5219577233054));
#92832=CARTESIAN_POINT('Ctrl Pts',(20.8130482446981,18.7784200373076,-15.5364346135072));
#92833=CARTESIAN_POINT('Ctrl Pts',(20.7724738455468,18.6158537801209,-15.5476702297927));
#92834=CARTESIAN_POINT('Ctrl Pts',(20.6924624647145,18.4050638743508,-15.5622010112452));
#92835=CARTESIAN_POINT('Ctrl Pts',(20.6694539963057,18.3512750079729,-15.565912287619));
#92836=CARTESIAN_POINT('Ctrl Pts',(20.6288110695379,18.2661919181628,-15.5717806675225));
#92837=CARTESIAN_POINT('Ctrl Pts',(20.6125580912548,18.2342753487285,-15.5739817853825));
#92838=CARTESIAN_POINT('Ctrl Pts',(20.5902741696631,18.193131774859,-15.5768207007394));
#92839=CARTESIAN_POINT('Ctrl Pts',(20.5849708416758,18.1835193592641,-15.5774840790439));
#92840=CARTESIAN_POINT('Ctrl Pts',(20.5761955106883,18.1679023061202,-15.5785621703011));
#92841=CARTESIAN_POINT('Ctrl Pts',(20.5727683978061,18.1618728010446,-15.5789784830163));
#92842=CARTESIAN_POINT('Ctrl Pts',(20.5661006471687,18.1502749061132,-15.579779464103));
#92843=CARTESIAN_POINT('Ctrl Pts',(20.5628641031591,18.1447042625287,-15.5801642743378));
#92844=CARTESIAN_POINT('Ctrl Pts',(20.5553663865783,18.1319339798337,-15.5810466685782));
#92845=CARTESIAN_POINT('Ctrl Pts',(20.5510878476226,18.1247446215906,-15.5815436155439));
#92846=CARTESIAN_POINT('Ctrl Pts',(20.5395434907498,18.1056053700408,-15.5828671818466));
#92847=CARTESIAN_POINT('Ctrl Pts',(20.5322016118998,18.0937016683609,-15.5836910170113));
#92848=CARTESIAN_POINT('Ctrl Pts',(20.4710613330323,17.9967362084341,-15.590409223576));
#92849=CARTESIAN_POINT('Ctrl Pts',(20.4113743223814,17.9155318379454,-15.5960735879851));
#92850=CARTESIAN_POINT('Ctrl Pts',(20.2350899268049,17.7084129682052,-15.6110568404912));
#92851=CARTESIAN_POINT('Ctrl Pts',(20.1086392270318,17.5919279864943,-15.6200635473757));
#92852=CARTESIAN_POINT('Ctrl Pts',(19.9371702672619,17.468685230952,-15.632094787001));
#92853=CARTESIAN_POINT('Ctrl Pts',(19.9041378002494,17.446331047384,-15.6344077557125));
#92854=CARTESIAN_POINT('Ctrl Pts',(19.8640122976131,17.4207988179777,-15.6372367510775));
#92855=CARTESIAN_POINT('Ctrl Pts',(19.8575059829887,17.416708394112,-15.6376960635362));
#92856=CARTESIAN_POINT('Ctrl Pts',(19.8474039941651,17.4104339102215,-15.6384103607666));
#92857=CARTESIAN_POINT('Ctrl Pts',(19.8438237620606,17.4082249407255,-15.6386637355539));
#92858=CARTESIAN_POINT('Ctrl Pts',(19.8372000634862,17.4041653901539,-15.6391329522938));
#92859=CARTESIAN_POINT('Ctrl Pts',(19.8341585013622,17.4023118127388,-15.6393485935521));
#92860=CARTESIAN_POINT('Ctrl Pts',(19.8273073388361,17.3981602783709,-15.6398347296075));
#92861=CARTESIAN_POINT('Ctrl Pts',(19.8234951890574,17.3958666644972,-15.6401055007096));
#92862=CARTESIAN_POINT('Ctrl Pts',(19.8137223624237,17.3900286347835,-15.6408002905011));
#92863=CARTESIAN_POINT('Ctrl Pts',(19.8077515007968,17.3865014923688,-15.6412253907565));
#92864=CARTESIAN_POINT('Ctrl Pts',(19.7727681064537,17.3660670996981,-15.6437191087663));
#92865=CARTESIAN_POINT('Ctrl Pts',(19.743375659397,17.3498237397996,-15.6458264339797));
#92866=CARTESIAN_POINT('Ctrl Pts',(19.6974282277872,17.3258399798626,-15.6491249626217));
#92867=CARTESIAN_POINT('Ctrl Pts',(19.6811369202531,17.3176025589441,-15.6502953209886));
#92868=CARTESIAN_POINT('Ctrl Pts',(19.6425584282783,17.2987184873438,-15.6530654176598));
#92869=CARTESIAN_POINT('Ctrl Pts',(19.6201875387926,17.2882492150893,-15.6546706773384));
#92870=CARTESIAN_POINT('Ctrl Pts',(19.5566270888549,17.2598486761793,-15.6592195096192));
#92871=CARTESIAN_POINT('Ctrl Pts',(19.5150429438074,17.2428337071169,-15.6621813147283));
#92872=CARTESIAN_POINT('Ctrl Pts',(19.3704830907159,17.188987511668,-15.6723715592087));
#92873=CARTESIAN_POINT('Ctrl Pts',(19.2652050271064,17.1588133823372,-15.6796015915757));
#92874=CARTESIAN_POINT('Ctrl Pts',(19.1041215716146,17.125878870974,-15.6901694287262));
#92875=CARTESIAN_POINT('Ctrl Pts',(19.0497690519771,17.1169582560398,-15.6936556299833));
#92876=CARTESIAN_POINT('Ctrl Pts',(18.961105536361,17.1059376743791,-15.699209071197));
#92877=CARTESIAN_POINT('Ctrl Pts',(18.9269852600988,17.1025358137451,-15.7013146787371));
#92878=CARTESIAN_POINT('Ctrl Pts',(18.882020100502,17.0991534568251,-15.7040498370852));
#92879=CARTESIAN_POINT('Ctrl Pts',(18.8712382299633,17.0984253984557,-15.7047026999878));
#92880=CARTESIAN_POINT('Ctrl Pts',(18.8535659125318,17.0973679203593,-15.7057680279105));
#92881=CARTESIAN_POINT('Ctrl Pts',(18.8466786918907,17.0969895720051,-15.7061820214219));
#92882=CARTESIAN_POINT('Ctrl Pts',(18.833340804196,17.0963222238964,-15.706981517379));
#92883=CARTESIAN_POINT('Ctrl Pts',(18.8268904305305,17.0960290636828,-15.7073671459535));
#92884=CARTESIAN_POINT('Ctrl Pts',(18.811989926927,17.0954201567187,-15.70825565166));
#92885=CARTESIAN_POINT('Ctrl Pts',(18.8035390085454,17.0951255161387,-15.7087578623163));
#92886=CARTESIAN_POINT('Ctrl Pts',(18.7807983227276,17.0944690557678,-15.7101047980134));
#92887=CARTESIAN_POINT('Ctrl Pts',(18.7665061253851,17.0942013114992,-15.7109465793941));
#92888=CARTESIAN_POINT('Ctrl Pts',(18.6350479161247,17.0930703660303,-15.718648079815));
#92889=CARTESIAN_POINT('Ctrl Pts',(18.5179952210324,17.1017905082359,-15.7251891697428));
#92890=CARTESIAN_POINT('Ctrl Pts',(18.2404051691153,17.145834873476,-15.7405740963719));
#92891=CARTESIAN_POINT('Ctrl Pts',(18.08210787952,17.1902161995463,-15.7492315175644));
#92892=CARTESIAN_POINT('Ctrl Pts',(17.901668165526,17.264237029948,-15.760446319959));
#92893=CARTESIAN_POINT('Ctrl Pts',(17.8730709881215,17.2767137367901,-15.7622678352236));
#92894=CARTESIAN_POINT('Ctrl Pts',(17.8382748814437,17.2928194544098,-15.764551266668));
#92895=CARTESIAN_POINT('Ctrl Pts',(17.8318034323742,17.2958547199911,-15.7649788385074));
#92896=CARTESIAN_POINT('Ctrl Pts',(17.8216539246104,17.3006779426256,-15.7656541737725));
#92897=CARTESIAN_POINT('Ctrl Pts',(17.8179653947633,17.3024439160643,-15.7659005957242));
#92898=CARTESIAN_POINT('Ctrl Pts',(17.8110620178731,17.3057736979643,-15.7663636981294));
#92899=CARTESIAN_POINT('Ctrl Pts',(17.8078460072386,17.3073349659571,-15.7665802207487));
#92900=CARTESIAN_POINT('Ctrl Pts',(17.800489613972,17.3109293078088,-15.7670772824539));
#92901=CARTESIAN_POINT('Ctrl Pts',(17.7963519234447,17.3129677664095,-15.7673581540515));
#92902=CARTESIAN_POINT('Ctrl Pts',(17.7855281696195,17.3183441853468,-15.768096212688));
#92903=CARTESIAN_POINT('Ctrl Pts',(17.7788531288448,17.321704020938,-15.7685547157601));
#92904=CARTESIAN_POINT('Ctrl Pts',(17.7341721533976,17.3444911856123,-15.77164558563));
#92905=CARTESIAN_POINT('Ctrl Pts',(17.696746216713,17.3650273842549,-15.7743405504313));
#92906=CARTESIAN_POINT('Ctrl Pts',(17.6537624983241,17.3903331382943,-15.7775396677328));
#92907=CARTESIAN_POINT('Ctrl Pts',(17.6475741898257,17.3940190319585,-15.7780028227472));
#92908=CARTESIAN_POINT('Ctrl Pts',(17.506733216783,17.4788837808983,-15.788601064497));
#92909=CARTESIAN_POINT('Ctrl Pts',(17.3815204068972,17.5747809998755,-15.7991743180983));
#92910=CARTESIAN_POINT('Ctrl Pts',(17.1996368765667,17.7493510037903,-15.8155534463536));
#92911=CARTESIAN_POINT('Ctrl Pts',(17.1356824256298,17.819571561161,-15.8215790722409));
#92912=CARTESIAN_POINT('Ctrl Pts',(17.063376756453,17.9105531859024,-15.8287171504957));
#92913=CARTESIAN_POINT('Ctrl Pts',(17.0503589587253,17.9274514677791,-15.8300171974182));
#92914=CARTESIAN_POINT('Ctrl Pts',(17.0322147377083,17.9517554217632,-15.8318514236441));
#92915=CARTESIAN_POINT('Ctrl Pts',(17.0268770682142,17.9590010836857,-15.8323938569715));
#92916=CARTESIAN_POINT('Ctrl Pts',(17.0177495690614,17.9715581794582,-15.833326444012));
#92917=CARTESIAN_POINT('Ctrl Pts',(17.013937824724,17.9768534597266,-15.833717444985));
#92918=CARTESIAN_POINT('Ctrl Pts',(17.0066870488709,17.9870250931465,-15.8344642231734));
#92919=CARTESIAN_POINT('Ctrl Pts',(17.003244040454,17.9918985221222,-15.8348201512138));
#92920=CARTESIAN_POINT('Ctrl Pts',(16.9943461593564,18.0046067587536,-15.8357434892715));
#92921=CARTESIAN_POINT('Ctrl Pts',(16.9889235577931,18.0124640793104,-15.8363096631929));
#92922=CARTESIAN_POINT('Ctrl Pts',(16.9706219355146,18.0393705675953,-15.8382327210528));
#92923=CARTESIAN_POINT('Ctrl Pts',(16.9579999147849,18.0585931779762,-15.839579912918));
#92924=CARTESIAN_POINT('Ctrl Pts',(16.8645247598485,18.2061350475879,-15.8497291248369));
#92925=CARTESIAN_POINT('Ctrl Pts',(16.7973961927158,18.3425421376678,-15.857987029616));
#92926=CARTESIAN_POINT('Ctrl Pts',(16.7454194505387,18.4848895412513,-15.8662164192772));
#92927=CARTESIAN_POINT('',(16.6170002518853,19.2099672937205,-14.8907771687908));
#92928=CARTESIAN_POINT('Ctrl Pts',(16.7454194503191,18.4848895418528,-15.6464962064494));
#92929=CARTESIAN_POINT('Ctrl Pts',(16.7464618212973,18.4820348265275,-15.646314727117));
#92930=CARTESIAN_POINT('Ctrl Pts',(16.7475103330494,18.4791823732292,-15.6461329005545));
#92931=CARTESIAN_POINT('Ctrl Pts',(16.7501831765914,18.4719590306671,-15.6456711873015));
#92932=CARTESIAN_POINT('Ctrl Pts',(16.7518158016389,18.4675912658523,-15.645390821652));
#92933=CARTESIAN_POINT('Ctrl Pts',(16.7547310336454,18.4598700180448,-15.6448930464087));
#92934=CARTESIAN_POINT('Ctrl Pts',(16.7560077574923,18.4565143610466,-15.6446759903617));
#92935=CARTESIAN_POINT('Ctrl Pts',(16.7587298590392,18.4494141674561,-15.6442151703432));
#92936=CARTESIAN_POINT('Ctrl Pts',(16.760177328531,18.4456705473598,-15.6439712873832));
#92937=CARTESIAN_POINT('Ctrl Pts',(16.7641078952561,18.4355901623563,-15.6433121688402));
#92938=CARTESIAN_POINT('Ctrl Pts',(16.7666108942137,18.429261281392,-15.6428957641459));
#92939=CARTESIAN_POINT('Ctrl Pts',(16.7791207398447,18.398070525457,-15.640831204365));
#92940=CARTESIAN_POINT('Ctrl Pts',(16.7895680677611,18.373389375823,-15.6391585768968));
#92941=CARTESIAN_POINT('Ctrl Pts',(16.8210382189566,18.3028068679415,-15.6342757171667));
#92942=CARTESIAN_POINT('Ctrl Pts',(16.8432373330588,18.2574522047139,-15.6310148787141));
#92943=CARTESIAN_POINT('Ctrl Pts',(16.9295816583965,18.0959373868848,-15.6190523488454));
#92944=CARTESIAN_POINT('Ctrl Pts',(17.002989257499,17.9850738644353,-15.6101841461185));
#92945=CARTESIAN_POINT('Ctrl Pts',(17.1511162430004,17.801451616154,-15.5948582198333));
#92946=CARTESIAN_POINT('Ctrl Pts',(17.2217357581854,17.7259377182922,-15.5883172744764));
#92947=CARTESIAN_POINT('Ctrl Pts',(17.3079107837369,17.6463416503839,-15.5811566207662));
#92948=CARTESIAN_POINT('Ctrl Pts',(17.3183213375557,17.6369160939192,-15.5803038124706));
#92949=CARTESIAN_POINT('Ctrl Pts',(17.3350950535145,17.6220304524294,-15.5789489199586));
#92950=CARTESIAN_POINT('Ctrl Pts',(17.3413980608891,17.6165034917723,-15.5784440350067));
#92951=CARTESIAN_POINT('Ctrl Pts',(17.3526049390447,17.6067935837632,-15.5775537343629));
#92952=CARTESIAN_POINT('Ctrl Pts',(17.3574953646643,17.6025953461111,-15.5771676859683));
#92953=CARTESIAN_POINT('Ctrl Pts',(17.3676821966819,17.5939308432624,-15.5763685838711));
#92954=CARTESIAN_POINT('Ctrl Pts',(17.3729815139306,17.5894681071075,-15.575955678056));
#92955=CARTESIAN_POINT('Ctrl Pts',(17.3867089330075,17.5780224830243,-15.5748932018281));
#92956=CARTESIAN_POINT('Ctrl Pts',(17.3951695181801,17.5710787403345,-15.5742452292214));
#92957=CARTESIAN_POINT('Ctrl Pts',(17.4313068150247,17.5418863312755,-15.5715060262037));
#92958=CARTESIAN_POINT('Ctrl Pts',(17.4594880963102,17.520269507589,-15.5694401343146));
#92959=CARTESIAN_POINT('Ctrl Pts',(17.5349316129331,17.4653584015064,-15.5640773301655));
#92960=CARTESIAN_POINT('Ctrl Pts',(17.5830375239335,17.4332723228912,-15.5608243484111));
#92961=CARTESIAN_POINT('Ctrl Pts',(17.770793085422,17.318862031781,-15.5486248546165));
#92962=CARTESIAN_POINT('Ctrl Pts',(17.918401471303,17.25070735247,-15.5400738399266));
#92963=CARTESIAN_POINT('Ctrl Pts',(18.0929193608975,17.1932848495841,-15.5298130893036));
#92964=CARTESIAN_POINT('Ctrl Pts',(18.113610929582,17.1868270419296,-15.5285934990093));
#92965=CARTESIAN_POINT('Ctrl Pts',(18.1746753193025,17.1687931780516,-15.5249758283697));
#92966=CARTESIAN_POINT('Ctrl Pts',(18.215295288226,17.1581001743488,-15.5225459138842));
#92967=CARTESIAN_POINT('Ctrl Pts',(18.2634485671725,17.1469443654395,-15.5196092826258));
#92968=CARTESIAN_POINT('Ctrl Pts',(18.2707026486073,17.1453040218832,-15.519165406912));
#92969=CARTESIAN_POINT('Ctrl Pts',(18.2824589271604,17.1427106496649,-15.5184434203876));
#92970=CARTESIAN_POINT('Ctrl Pts',(18.2869559243674,17.1417340019477,-15.5181666274569));
#92971=CARTESIAN_POINT('Ctrl Pts',(18.2949509737732,17.1400249336552,-15.5176733698364));
#92972=CARTESIAN_POINT('Ctrl Pts',(18.2984477327466,17.1392867005484,-15.5174572411903));
#92973=CARTESIAN_POINT('Ctrl Pts',(18.3059565647136,17.1377212927563,-15.5169922697591));
#92974=CARTESIAN_POINT('Ctrl Pts',(18.3099691142896,17.1368969197004,-15.5167432765022));
#92975=CARTESIAN_POINT('Ctrl Pts',(18.3210204168516,17.1346598535017,-15.5160561123951));
#92976=CARTESIAN_POINT('Ctrl Pts',(18.3280639262587,17.1332713264984,-15.5156165998363));
#92977=CARTESIAN_POINT('Ctrl Pts',(18.3661847547162,17.1259575888047,-15.5132300022163));
#92978=CARTESIAN_POINT('Ctrl Pts',(18.39738310792,17.1206941060276,-15.5112485866999));
#92979=CARTESIAN_POINT('Ctrl Pts',(18.5904484628164,17.0925559980764,-15.498861442055));
#92980=CARTESIAN_POINT('Ctrl Pts',(18.7543927490247,17.0877958224382,-15.487851091797));
#92981=CARTESIAN_POINT('Ctrl Pts',(19.0338618281357,17.1120781888918,-15.4695259696804));
#92982=CARTESIAN_POINT('Ctrl Pts',(19.1494465050029,17.1318650985331,-15.4620691886714));
#92983=CARTESIAN_POINT('Ctrl Pts',(19.2766584375527,17.1646825527341,-15.4540472965382));
#92984=CARTESIAN_POINT('Ctrl Pts',(19.2904615651038,17.1683928872342,-15.4531791278567));
#92985=CARTESIAN_POINT('Ctrl Pts',(19.3123692432902,17.1745203137437,-15.4518045729043));
#92986=CARTESIAN_POINT('Ctrl Pts',(19.3204985291414,17.17684662017,-15.4512952569314));
#92987=CARTESIAN_POINT('Ctrl Pts',(19.3348106926231,17.1810351720397,-15.4503998144226));
#92988=CARTESIAN_POINT('Ctrl Pts',(19.3409993555557,17.1828771055693,-15.4500130314626));
#92989=CARTESIAN_POINT('Ctrl Pts',(19.3537815603101,17.1867452246307,-15.4492149750924));
#92990=CARTESIAN_POINT('Ctrl Pts',(19.3603738276835,17.1887753814597,-15.4488038369074));
#92991=CARTESIAN_POINT('Ctrl Pts',(19.3772687438688,17.1940688872014,-15.447751247656));
#92992=CARTESIAN_POINT('Ctrl Pts',(19.3875566202858,17.1973789976141,-15.4471113371985));
#92993=CARTESIAN_POINT('Ctrl Pts',(19.4303799581408,17.2115201194859,-15.4444516272409));
#92994=CARTESIAN_POINT('Ctrl Pts',(19.462676268386,17.2230623925964,-15.4424553349185));
#92995=CARTESIAN_POINT('Ctrl Pts',(19.5460739539732,17.2551733482917,-15.4373138962826));
#92996=CARTESIAN_POINT('Ctrl Pts',(19.5966791462783,17.2769608759741,-15.434208085989));
#92997=CARTESIAN_POINT('Ctrl Pts',(19.7450258090312,17.3478127900661,-15.4250667264352));
#92998=CARTESIAN_POINT('Ctrl Pts',(19.8398767814879,17.4024986323835,-15.4191799166778));
#92999=CARTESIAN_POINT('Ctrl Pts',(19.9655432814717,17.4885489782426,-15.4108879396568));
#93000=CARTESIAN_POINT('Ctrl Pts',(20.0002583105075,17.513906579616,-15.4085384339124));
#93001=CARTESIAN_POINT('Ctrl Pts',(20.0938032272092,17.5867054555196,-15.4019765558035));
#93002=CARTESIAN_POINT('Ctrl Pts',(20.1508965821154,17.6362622166131,-15.3977073634541));
#93003=CARTESIAN_POINT('Ctrl Pts',(20.2120392756548,17.6953552427986,-15.3926678160888));
#93004=CARTESIAN_POINT('Ctrl Pts',(20.2188211823139,17.7019986151866,-15.3921019251866));
#93005=CARTESIAN_POINT('Ctrl Pts',(20.2288083534064,17.7119142902945,-15.3912578545929));
#93006=CARTESIAN_POINT('Ctrl Pts',(20.2320481580851,17.7151518480775,-15.3909823451046));
#93007=CARTESIAN_POINT('Ctrl Pts',(20.2377957106074,17.7209328140889,-15.3904904946403));
#93008=CARTESIAN_POINT('Ctrl Pts',(20.2403075532293,17.7234720800524,-15.390274482435));
#93009=CARTESIAN_POINT('Ctrl Pts',(20.2456963664194,17.7289473719113,-15.3898087570877));
#93010=CARTESIAN_POINT('Ctrl Pts',(20.248571173344,17.7318853807491,-15.3895588881872));
#93011=CARTESIAN_POINT('Ctrl Pts',(20.2564882266924,17.7400237703792,-15.3888668918282));
#93012=CARTESIAN_POINT('Ctrl Pts',(20.2615123118425,17.7452416289841,-15.388423391894));
#93013=CARTESIAN_POINT('Ctrl Pts',(20.2889763366229,17.7740594634095,-15.3859754195532));
#93014=CARTESIAN_POINT('Ctrl Pts',(20.3108948923896,17.7981476575058,-15.3839345405864));
#93015=CARTESIAN_POINT('Ctrl Pts',(20.4389281604584,17.9455461493966,-15.3715279086093));
#93016=CARTESIAN_POINT('Ctrl Pts',(20.5310941831851,18.0802454240744,-15.3605727162411));
#93017=CARTESIAN_POINT('Ctrl Pts',(20.6613730595803,18.3275042306929,-15.3423172746963));
#93018=CARTESIAN_POINT('Ctrl Pts',(20.7071813425255,18.4351811557761,-15.3348770814132));
#93019=CARTESIAN_POINT('Ctrl Pts',(20.7483642049038,18.5596705659051,-15.326870626374));
#93020=CARTESIAN_POINT('Ctrl Pts',(20.7527146990851,18.5732820677364,-15.326002658254));
#93021=CARTESIAN_POINT('Ctrl Pts',(20.75941939604,18.595015626581,-15.3246283598287));
#93022=CARTESIAN_POINT('Ctrl Pts',(20.7618632718003,18.6031093582938,-15.3241191015222));
#93023=CARTESIAN_POINT('Ctrl Pts',(20.7660879209759,18.6174097620832,-15.3232237260909));
#93024=CARTESIAN_POINT('Ctrl Pts',(20.7678888955056,18.623610307123,-15.3228369528513));
#93025=CARTESIAN_POINT('Ctrl Pts',(20.771555220673,18.6364520854575,-15.3220388836862));
#93026=CARTESIAN_POINT('Ctrl Pts',(20.7734165372754,18.6430943981465,-15.3216277231476));
#93027=CARTESIAN_POINT('Ctrl Pts',(20.7781109545724,18.6601676899669,-15.3205750086698));
#93028=CARTESIAN_POINT('Ctrl Pts',(20.7808967179971,18.6706115648992,-15.3199349960594));
#93029=CARTESIAN_POINT('Ctrl Pts',(20.7921897540702,18.714290006212,-15.3172742934018));
#93030=CARTESIAN_POINT('Ctrl Pts',(20.7999688282541,18.7477086456871,-15.3152771329364));
#93031=CARTESIAN_POINT('Ctrl Pts',(20.8181177594599,18.8352622375545,-15.3101329530553));
#93032=CARTESIAN_POINT('Ctrl Pts',(20.8271923252784,18.8896400207663,-15.3070253246903));
#93033=CARTESIAN_POINT('Ctrl Pts',(20.847909952043,19.0527894438711,-15.2978807931925));
#93034=CARTESIAN_POINT('Ctrl Pts',(20.8532599351002,19.1621729953013,-15.291992619048));
#93035=CARTESIAN_POINT('Ctrl Pts',(20.8488264518945,19.3172966006862,-15.2835435861459));
#93036=CARTESIAN_POINT('Ctrl Pts',(20.846029397009,19.3630574755655,-15.2810373712711));
#93037=CARTESIAN_POINT('Ctrl Pts',(20.8396445266059,19.4311322580234,-15.2772457677915));
#93038=CARTESIAN_POINT('Ctrl Pts',(20.837181382164,19.4535388773749,-15.2759874359774));
#93039=CARTESIAN_POINT('Ctrl Pts',(20.8335686285498,19.4821838340803,-15.2743608706973));
#93040=CARTESIAN_POINT('Ctrl Pts',(20.8327480887147,19.4884627121551,-15.2740032275575));
#93041=CARTESIAN_POINT('Ctrl Pts',(20.8258132327739,19.5397376289191,-15.2710729163464));
#93042=CARTESIAN_POINT('Ctrl Pts',(20.8182812484857,19.5845265046774,-15.2684522282174));
#93043=CARTESIAN_POINT('Ctrl Pts',(20.8078132896979,19.6364942294351,-15.2653039568065));
#93044=CARTESIAN_POINT('Ctrl Pts',(20.8062705546122,19.6439453133609,-15.264849955684));
#93045=CARTESIAN_POINT('Ctrl Pts',(20.8037300105769,19.6558908609339,-15.2641176824912));
#93046=CARTESIAN_POINT('Ctrl Pts',(20.8027576347759,19.6603907458598,-15.2638408259588));
#93047=CARTESIAN_POINT('Ctrl Pts',(20.8010024651387,19.6683867562725,-15.2633470156382));
#93048=CARTESIAN_POINT('Ctrl Pts',(20.8002254661125,19.6718841055093,-15.2631303959459));
#93049=CARTESIAN_POINT('Ctrl Pts',(20.7985516858265,19.679328645847,-15.2626679244081));
#93050=CARTESIAN_POINT('Ctrl Pts',(20.7976524747891,19.6832751810458,-15.2624219404899));
#93051=CARTESIAN_POINT('Ctrl Pts',(20.7951765541253,19.6939996263973,-15.2617513204872));
#93052=CARTESIAN_POINT('Ctrl Pts',(20.7935777498196,19.7007723100772,-15.2613254457314));
#93053=CARTESIAN_POINT('Ctrl Pts',(20.7852192197669,19.7354150545794,-15.259135373659));
#93054=CARTESIAN_POINT('Ctrl Pts',(20.7779274186208,19.7631521130403,-15.2573430682459));
#93055=CARTESIAN_POINT('Ctrl Pts',(20.7547774541449,19.8444571910483,-15.251991425533));
#93056=CARTESIAN_POINT('Ctrl Pts',(20.7373604286853,19.8975534703494,-15.248370238316));
#93057=CARTESIAN_POINT('Ctrl Pts',(20.6691425351427,20.0807123067221,-15.2355657320242));
#93058=CARTESIAN_POINT('Ctrl Pts',(20.6075942740134,20.2064022750081,-15.2262394981157));
#93059=CARTESIAN_POINT('Ctrl Pts',(20.4870741947634,20.4011306239625,-15.2114604455813));
#93060=CARTESIAN_POINT('Ctrl Pts',(20.4352576128017,20.4740938961757,-15.2058281269232));
#93061=CARTESIAN_POINT('Ctrl Pts',(20.3703515631348,20.5542163906147,-15.1995368715949));
#93062=CARTESIAN_POINT('Ctrl Pts',(20.3616241760003,20.5647785142856,-15.1987051182947));
#93063=CARTESIAN_POINT('Ctrl Pts',(20.3474571411605,20.5815887988599,-15.1973772297129));
#93064=CARTESIAN_POINT('Ctrl Pts',(20.3420823980459,20.5878909201756,-15.1968784662085));
#93065=CARTESIAN_POINT('Ctrl Pts',(20.3324697868567,20.5990290640551,-15.1959952251807));
#93066=CARTESIAN_POINT('Ctrl Pts',(20.3282466369264,20.6038775984337,-15.1956101475697));
#93067=CARTESIAN_POINT('Ctrl Pts',(20.3193976977879,20.6139439623226,-15.1948093789898));
#93068=CARTESIAN_POINT('Ctrl Pts',(20.3147680808237,20.6191583355595,-15.1943938541769));
#93069=CARTESIAN_POINT('Ctrl Pts',(20.3026698665308,20.6326497938427,-15.1933167766899));
#93070=CARTESIAN_POINT('Ctrl Pts',(20.2951614388007,20.6408909943367,-15.1926569076469));
#93071=CARTESIAN_POINT('Ctrl Pts',(20.2621921186869,20.676508628919,-15.1897959849049));
#93072=CARTESIAN_POINT('Ctrl Pts',(20.2360727348287,20.7032682213898,-15.1876232211937));
#93073=CARTESIAN_POINT('Ctrl Pts',(20.1647139335123,20.772602979298,-15.1819140029514));
#93074=CARTESIAN_POINT('Ctrl Pts',(20.1182857599495,20.8139036243126,-15.1784292939751));
#93075=CARTESIAN_POINT('Ctrl Pts',(19.9653800727645,20.9383159583459,-15.1675264745593));
#93076=CARTESIAN_POINT('Ctrl Pts',(19.8527475927383,21.0133095243525,-15.1603353968679));
#93077=CARTESIAN_POINT('Ctrl Pts',(19.6615335535597,21.1157523342815,-15.1483693533313));
#93078=CARTESIAN_POINT('Ctrl Pts',(19.5871469487989,21.150210420812,-15.1437602921818));
#93079=CARTESIAN_POINT('Ctrl Pts',(19.5020345749563,21.1837909118349,-15.1383386088654));
#93080=CARTESIAN_POINT('Ctrl Pts',(19.4930842240697,21.1872520646618,-15.1377666780148));
#93081=CARTESIAN_POINT('Ctrl Pts',(19.4798089805932,21.1922821927852,-15.1369153079885));
#93082=CARTESIAN_POINT('Ctrl Pts',(19.4755018636163,21.1938981689231,-15.1366386065038));
#93083=CARTESIAN_POINT('Ctrl Pts',(19.4678394783845,21.1967445434177,-15.1361454493929));
#93084=CARTESIAN_POINT('Ctrl Pts',(19.4644863269233,21.197980497566,-15.1359293292924));
#93085=CARTESIAN_POINT('Ctrl Pts',(19.4572819031519,21.2006153088292,-15.1354643052791));
#93086=CARTESIAN_POINT('Ctrl Pts',(19.453429751928,21.2020114565059,-15.1352152505222));
#93087=CARTESIAN_POINT('Ctrl Pts',(19.442812772387,21.2058245683849,-15.134527747316));
#93088=CARTESIAN_POINT('Ctrl Pts',(19.4360397305469,21.2082182700584,-15.134087955009));
#93089=CARTESIAN_POINT('Ctrl Pts',(19.3993117870122,21.2209886069406,-15.1316971125447));
#93090=CARTESIAN_POINT('Ctrl Pts',(19.3691405599911,21.2307252765818,-15.1297115903816));
#93091=CARTESIAN_POINT('Ctrl Pts',(19.1821576219572,21.2864634780219,-15.1173231378092));
#93092=CARTESIAN_POINT('Ctrl Pts',(19.020677317936,21.3148559450112,-15.1063166472014));
#93093=CARTESIAN_POINT('Ctrl Pts',(18.7407053511653,21.3312219271883,-15.0879963471976));
#93094=CARTESIAN_POINT('Ctrl Pts',(18.6234911258319,21.3283525024668,-15.0805406775329));
#93095=CARTESIAN_POINT('Ctrl Pts',(18.4928879276334,21.3142732198246,-15.0725198193826));
#93096=CARTESIAN_POINT('Ctrl Pts',(18.4786936111983,21.3125974715049,-15.0716516639673));
#93097=CARTESIAN_POINT('Ctrl Pts',(18.4561305025961,21.3097017500052,-15.0702771259826));
#93098=CARTESIAN_POINT('Ctrl Pts',(18.4477503608139,21.3085751811004,-15.0697678138239));
#93099=CARTESIAN_POINT('Ctrl Pts',(18.4329830758618,21.306499821612,-15.0688723757521));
#93100=CARTESIAN_POINT('Ctrl Pts',(18.4265931448461,21.3055719653025,-15.0684855934351));
#93101=CARTESIAN_POINT('Ctrl Pts',(18.4133859842095,21.3035924666151,-15.0676875362193));
#93102=CARTESIAN_POINT('Ctrl Pts',(18.4065694415479,21.302536710072,-15.0672763965563));
#93103=CARTESIAN_POINT('Ctrl Pts',(18.3890865791447,21.299741373465,-15.0662237990248));
#93104=CARTESIAN_POINT('Ctrl Pts',(18.3784281163115,21.2979533859664,-15.0655838818129));
#93105=CARTESIAN_POINT('Ctrl Pts',(18.3340091343197,21.2901518018149,-15.0629241062285));
#93106=CARTESIAN_POINT('Ctrl Pts',(18.3003824320171,21.2833997946169,-15.0609277565146));
#93107=CARTESIAN_POINT('Ctrl Pts',(18.213215384097,21.2636825440875,-15.0557861366747));
#93108=CARTESIAN_POINT('Ctrl Pts',(18.1599898267852,21.2494394051595,-15.0526802062049));
#93109=CARTESIAN_POINT('Ctrl Pts',(18.0045375861835,21.2012676129357,-15.0436307844694));
#93110=CARTESIAN_POINT('Ctrl Pts',(17.9042759436445,21.1615997755708,-15.0378298283945));
#93111=CARTESIAN_POINT('Ctrl Pts',(17.6993597569857,21.0618551640889,-15.0254260779334));
#93112=CARTESIAN_POINT('Ctrl Pts',(17.5959470071513,21.0001261074266,-15.018828609812));
#93113=CARTESIAN_POINT('Ctrl Pts',(17.4906331647077,20.9244229396325,-15.0111418568529));
#93114=CARTESIAN_POINT('Ctrl Pts',(17.4829565968111,20.9188260019371,-15.0105755732857));
#93115=CARTESIAN_POINT('Ctrl Pts',(17.4716343320212,20.9104537095105,-15.0097310279634));
#93116=CARTESIAN_POINT('Ctrl Pts',(17.4679594328788,20.9077177938474,-15.0094554407745));
#93117=CARTESIAN_POINT('Ctrl Pts',(17.4615604000717,20.9029214316605,-15.0089729368512));
#93118=CARTESIAN_POINT('Ctrl Pts',(17.4588323369226,20.9008662956718,-15.0087663928243));
#93119=CARTESIAN_POINT('Ctrl Pts',(17.4529434263976,20.8964076132299,-15.0083187005526));
#93120=CARTESIAN_POINT('Ctrl Pts',(17.4497844117452,20.894001809205,-15.0080773970113));
#93121=CARTESIAN_POINT('Ctrl Pts',(17.4413944510692,20.8875749094958,-15.0074335099071));
#93122=CARTESIAN_POINT('Ctrl Pts',(17.4361755526817,20.8835382607191,-15.0070298524683));
#93123=CARTESIAN_POINT('Ctrl Pts',(17.4245779490864,20.8744809250067,-15.0061259807316));
#93124=CARTESIAN_POINT('Ctrl Pts',(17.4182091124819,20.8694478378671,-15.0056249515416));
#93125=CARTESIAN_POINT('Ctrl Pts',(17.398985283648,20.8540754273455,-15.0040988253626));
#93126=CARTESIAN_POINT('Ctrl Pts',(17.3862223578311,20.8436225971152,-15.0030667181486));
#93127=CARTESIAN_POINT('Ctrl Pts',(17.3390418057299,20.8040514883759,-14.9991842510155));
#93128=CARTESIAN_POINT('Ctrl Pts',(17.3054366293051,20.7739867513939,-14.9962835432857));
#93129=CARTESIAN_POINT('Ctrl Pts',(17.2178827406146,20.6904733250081,-14.9884085533946));
#93130=CARTESIAN_POINT('Ctrl Pts',(17.1658065505382,20.6351564430838,-14.9833805822346));
#93131=CARTESIAN_POINT('Ctrl Pts',(17.0169228477852,20.4589166570284,-14.9681407804334));
#93132=CARTESIAN_POINT('Ctrl Pts',(16.9302834974346,20.3300500983987,-14.9580559665156));
#93133=CARTESIAN_POINT('Ctrl Pts',(16.8473598005248,20.1716514176227,-14.9470407174499));
#93134=CARTESIAN_POINT('Ctrl Pts',(16.8366142451859,20.150249572677,-14.9455780297531));
#93135=CARTESIAN_POINT('Ctrl Pts',(16.8220268810556,20.1199235275425,-14.9435403653674));
#93136=CARTESIAN_POINT('Ctrl Pts',(16.8178801418033,20.1111488101519,-14.9429548210001));
#93137=CARTESIAN_POINT('Ctrl Pts',(16.8112693178155,20.0969072605944,-14.9420109076378));
#93138=CARTESIAN_POINT('Ctrl Pts',(16.8087678968943,20.0914580063287,-14.9416512510367));
#93139=CARTESIAN_POINT('Ctrl Pts',(16.8036027081718,20.0800785676884,-14.9409033144092));
#93140=CARTESIAN_POINT('Ctrl Pts',(16.800943033911,20.0741465857094,-14.9405151783309));
#93141=CARTESIAN_POINT('Ctrl Pts',(16.7947203277592,20.0600947984488,-14.9395998476362));
#93142=CARTESIAN_POINT('Ctrl Pts',(16.7911808847732,20.0519646324747,-14.9390734650396));
#93143=CARTESIAN_POINT('Ctrl Pts',(16.7796053595027,20.0249122838459,-14.9373324251423));
#93144=CARTESIAN_POINT('Ctrl Pts',(16.7717936629083,20.0058949309126,-14.9361253930586));
#93145=CARTESIAN_POINT('Ctrl Pts',(16.7318169225117,19.9043904128562,-14.9297674203842));
#93146=CARTESIAN_POINT('Ctrl Pts',(16.7045711712959,19.8200554557607,-14.9247836505034));
#93147=CARTESIAN_POINT('Ctrl Pts',(16.6389736836006,19.5628932602865,-14.9101349610871));
#93148=CARTESIAN_POINT('Ctrl Pts',(16.6169140089545,19.3867612829644,-14.9008598344646));
#93149=CARTESIAN_POINT('Ctrl Pts',(16.6170002518853,19.2099672937205,-14.8907771687908));
#93150=CARTESIAN_POINT('Ctrl Pts',(16.6170002532686,19.2099644618986,-14.8907770072903));
#93151=CARTESIAN_POINT('Ctrl Pts',(16.6170133611387,19.1831674202198,-14.8892487548365));
#93152=CARTESIAN_POINT('Ctrl Pts',(16.6175352642807,19.1563740130565,-14.8877018056538));
#93153=CARTESIAN_POINT('Ctrl Pts',(16.6191227654004,19.1151184461241,-14.8852809873123));
#93154=CARTESIAN_POINT('Ctrl Pts',(16.6198286097268,19.1006446791055,-14.8844242999335));
#93155=CARTESIAN_POINT('Ctrl Pts',(16.6209600190457,19.0814889215016,-14.8832793662802));
#93156=CARTESIAN_POINT('Ctrl Pts',(16.6212526903932,19.076799085809,-14.8829981723266));
#93157=CARTESIAN_POINT('Ctrl Pts',(16.6217938179286,19.068568820797,-14.8825030883143));
#93158=CARTESIAN_POINT('Ctrl Pts',(16.6220355693794,19.0650279486961,-14.8822895662434));
#93159=CARTESIAN_POINT('Ctrl Pts',(16.6225281743401,19.0580703880282,-14.8818689511269));
#93160=CARTESIAN_POINT('Ctrl Pts',(16.6227784202666,19.0546536603399,-14.8816618916634));
#93161=CARTESIAN_POINT('Ctrl Pts',(16.6233330673747,19.0473250324884,-14.8812166617965));
#93162=CARTESIAN_POINT('Ctrl Pts',(16.6236400494779,19.0434133832307,-14.8809783504605));
#93163=CARTESIAN_POINT('Ctrl Pts',(16.6244765273423,19.0331216587381,-14.8803496189784));
#93164=CARTESIAN_POINT('Ctrl Pts',(16.6250240881385,19.0267431500854,-14.8799582055379));
#93165=CARTESIAN_POINT('Ctrl Pts',(16.6274167961225,19.0002797749452,-14.8783273302293));
#93166=CARTESIAN_POINT('Ctrl Pts',(16.629519932923,18.9802200469978,-14.8770744361996));
#93167=CARTESIAN_POINT('Ctrl Pts',(16.6324142606819,18.9559616685905,-14.8755415586506));
#93168=CARTESIAN_POINT('Ctrl Pts',(16.6329320450474,18.9517306067433,-14.8752735437659));
#93169=CARTESIAN_POINT('Ctrl Pts',(16.6366907711341,18.9217671159181,-14.8733710044627));
#93170=CARTESIAN_POINT('Ctrl Pts',(16.6403914470368,18.8960956066903,-14.8717174084526));
#93171=CARTESIAN_POINT('Ctrl Pts',(16.665994580413,18.7389851978773,-14.8614773061057));
#93172=CARTESIAN_POINT('Ctrl Pts',(16.6997789097244,18.6098841517055,-14.8525677443131));
#93173=CARTESIAN_POINT('Ctrl Pts',(16.7454194448477,18.4848895568371,-14.8438385225655));
#93174=CARTESIAN_POINT('Origin',(18.734,19.211,0.));
#93175=CARTESIAN_POINT('',(16.7454194461219,18.4848895533475,-14.0426552599844));
#93176=CARTESIAN_POINT('',(16.7454194503191,18.4848895418526,-14.2664527091109));
#93177=CARTESIAN_POINT('',(16.7454194503191,18.4848895418526,0.));
#93178=CARTESIAN_POINT('',(16.6195738484597,19.2114672066323,-14.3109440134334));
#93179=CARTESIAN_POINT('Ctrl Pts',(16.7454194503191,18.4848895418526,-14.2664527091109));
#93180=CARTESIAN_POINT('Ctrl Pts',(16.7196506946332,18.5554617885013,-14.270975824323));
#93181=CARTESIAN_POINT('Ctrl Pts',(16.6976093487813,18.627498828733,-14.2754989395351));
#93182=CARTESIAN_POINT('Ctrl Pts',(16.6794520907032,18.7005865515055,-14.2800220547472));
#93183=CARTESIAN_POINT('Ctrl Pts',(16.6613181210866,18.7735805321165,-14.2845393686211));
#93184=CARTESIAN_POINT('Ctrl Pts',(16.6470584426659,18.8476220952149,-14.289056682495));
#93185=CARTESIAN_POINT('Ctrl Pts',(16.6367803549673,18.922280827639,-14.2935739963689));
#93186=CARTESIAN_POINT('Ctrl Pts',(16.6265157659132,18.9968415076116,-14.2980853774646));
#93187=CARTESIAN_POINT('Ctrl Pts',(16.6202224201554,19.072017312509,-14.3025967585603));
#93188=CARTESIAN_POINT('Ctrl Pts',(16.6179565327787,19.1473678946593,-14.3071081396561));
#93189=CARTESIAN_POINT('Ctrl Pts',(16.61731437944,19.1687222781118,-14.3083866667632));
#93190=CARTESIAN_POINT('Ctrl Pts',(16.6169953775011,19.1900906491545,-14.3096651938704));
#93191=CARTESIAN_POINT('Ctrl Pts',(16.617000050606,19.2114628884564,-14.3109437209775));
#93192=CARTESIAN_POINT('Ctrl Pts',(16.6203928462353,19.2114685807016,-14.3109441064946));
#93193=CARTESIAN_POINT('Ctrl Pts',(16.6197599964399,19.5369558005646,-14.3304466040344));
#93194=CARTESIAN_POINT('Ctrl Pts',(16.8436652507848,20.5691167836237,-14.3923410371346));
#93195=CARTESIAN_POINT('Ctrl Pts',(18.453125516026,21.6984565773647,-14.4966274057954));
#93196=CARTESIAN_POINT('Ctrl Pts',(20.6735253020556,20.7935840586526,-14.6238032124768));
#93197=CARTESIAN_POINT('Ctrl Pts',(21.114531003966,18.4367888923735,-14.7509790191583));
#93198=CARTESIAN_POINT('Ctrl Pts',(19.3715472621554,16.7902843643798,-14.8781548258396));
#93199=CARTESIAN_POINT('Ctrl Pts',(17.4471161436709,17.2650914732991,-14.9832889524729));
#93200=CARTESIAN_POINT('Ctrl Pts',(16.8648290097867,18.166885156152,-15.0460311435457));
#93201=CARTESIAN_POINT('Ctrl Pts',(16.7486736478041,18.4860706551708,-15.066381399058));
#93202=CARTESIAN_POINT('Ctrl Pts',(16.7454194448477,18.484889556837,-14.8438385225655));
#93203=CARTESIAN_POINT('Ctrl Pts',(16.760364385294,18.4439602212943,-14.840980148999));
#93204=CARTESIAN_POINT('Ctrl Pts',(16.7765805848748,18.4034713560533,-14.838138763469));
#93205=CARTESIAN_POINT('Ctrl Pts',(16.8176683039001,18.3094224023408,-14.8315216662765));
#93206=CARTESIAN_POINT('Ctrl Pts',(16.8435369451236,18.2563693039662,-14.8277760980566));
#93207=CARTESIAN_POINT('Ctrl Pts',(16.8887243955929,18.1727583809304,-14.8218600131763));
#93208=CARTESIAN_POINT('Ctrl Pts',(16.9066661974489,18.1414958436656,-14.8196445879183));
#93209=CARTESIAN_POINT('Ctrl Pts',(16.9311171312812,18.1013048027343,-14.8167901761693));
#93210=CARTESIAN_POINT('Ctrl Pts',(16.9369092150479,18.0919491580119,-14.8161252602874));
#93211=CARTESIAN_POINT('Ctrl Pts',(16.9464735387144,18.0767661944531,-14.8150453023116));
#93212=CARTESIAN_POINT('Ctrl Pts',(16.9502019067965,18.0709116087291,-14.8146286499345));
#93213=CARTESIAN_POINT('Ctrl Pts',(16.957445284155,18.05965998839,-14.8138274432605));
#93214=CARTESIAN_POINT('Ctrl Pts',(16.9609562569011,18.054260458358,-14.8134427448301));
#93215=CARTESIAN_POINT('Ctrl Pts',(16.9690774063331,18.0418947793422,-14.8125612071051));
#93216=CARTESIAN_POINT('Ctrl Pts',(16.9737043014657,18.0349396973884,-14.8120650007214));
#93217=CARTESIAN_POINT('Ctrl Pts',(16.9861630821549,18.0164500909454,-14.8107447111344));
#93218=CARTESIAN_POINT('Ctrl Pts',(16.9940680310008,18.0049651191932,-14.8099233900928));
#93219=CARTESIAN_POINT('Ctrl Pts',(17.0584934135661,17.9133145097415,-14.8033573529328));
#93220=CARTESIAN_POINT('Ctrl Pts',(17.1204130387034,17.8370820292176,-14.7978303323002));
#93221=CARTESIAN_POINT('Ctrl Pts',(17.2808171221161,17.6654700582512,-14.7848750373219));
#93222=CARTESIAN_POINT('Ctrl Pts',(17.3836930602115,17.5748239666527,-14.7775970535287));
#93223=CARTESIAN_POINT('Ctrl Pts',(17.5362188245962,17.464676453206,-14.7671723063572));
#93224=CARTESIAN_POINT('Ctrl Pts',(17.57892459575,17.4361406322258,-14.764285394078));
#93225=CARTESIAN_POINT('Ctrl Pts',(17.6379507252786,17.3997326701052,-14.7602785698418));
#93226=CARTESIAN_POINT('Ctrl Pts',(17.6533986661325,17.3904742335635,-14.7592284235887));
#93227=CARTESIAN_POINT('Ctrl Pts',(17.6764327302698,17.3770656532769,-14.7576575044492));
#93228=CARTESIAN_POINT('Ctrl Pts',(17.6839295734656,17.3727628520983,-14.7571454373302));
#93229=CARTESIAN_POINT('Ctrl Pts',(17.6975506155132,17.3650555891748,-14.7562132581507));
#93230=CARTESIAN_POINT('Ctrl Pts',(17.7036658083792,17.361635367238,-14.7557941025942));
#93231=CARTESIAN_POINT('Ctrl Pts',(17.7133275446521,17.3562943614642,-14.7551306506557));
#93232=CARTESIAN_POINT('Ctrl Pts',(17.7168628546947,17.354353212445,-14.7548876354203));
#93233=CARTESIAN_POINT('Ctrl Pts',(17.7204127490508,17.352417237565,-14.7546433429248));
#93234=CARTESIAN_POINT('Ctrl Pts',(17.7204218420691,17.3524122786716,-14.7546427171702));
#93235=CARTESIAN_POINT('Ctrl Pts',(17.7204400832236,17.3524023309998,-14.7546414618645));
#93236=CARTESIAN_POINT('Ctrl Pts',(17.7204492316218,17.3523973420797,-14.7546408322952));
#93237=CARTESIAN_POINT('Ctrl Pts',(17.7204675838462,17.3523873341884,-14.7546395693386));
#93238=CARTESIAN_POINT('Ctrl Pts',(17.7204767880041,17.3523823150375,-14.7546389359284));
#93239=CARTESIAN_POINT('Ctrl Pts',(17.7204952526121,17.3523722462167,-14.7546376652303));
#93240=CARTESIAN_POINT('Ctrl Pts',(17.7205045126594,17.3523671967676,-14.7546370279702));
#93241=CARTESIAN_POINT('Ctrl Pts',(17.7205230894845,17.3523570671147,-14.7546357495421));
#93242=CARTESIAN_POINT('Ctrl Pts',(17.7205324061711,17.3523519869617,-14.7546351083804));
#93243=CARTESIAN_POINT('Ctrl Pts',(17.7205510966092,17.352341795722,-14.7546338221261));
#93244=CARTESIAN_POINT('Ctrl Pts',(17.7205604702178,17.3523366847143,-14.7546331770432));
#93245=CARTESIAN_POINT('Ctrl Pts',(17.7205792745839,17.3523264317228,-14.7546318829408));
#93246=CARTESIAN_POINT('Ctrl Pts',(17.7205887057091,17.3523212895395,-14.7546312338958));
#93247=CARTESIAN_POINT('Ctrl Pts',(17.7206076260477,17.3523109736881,-14.7546299318044));
#93248=CARTESIAN_POINT('Ctrl Pts',(17.7206171145797,17.3523058003926,-14.7546292788048));
#93249=CARTESIAN_POINT('Ctrl Pts',(17.7206361498426,17.3522954222598,-14.7546279687965));
#93250=CARTESIAN_POINT('Ctrl Pts',(17.720645696871,17.3522902172614,-14.7546273117672));
#93251=CARTESIAN_POINT('Ctrl Pts',(17.7206648494162,17.3522797755684,-14.7546259936795));
#93252=CARTESIAN_POINT('Ctrl Pts',(17.7206744549312,17.352274538876,-14.7546253326212));
#93253=CARTESIAN_POINT('Ctrl Pts',(17.7206937248093,17.3522640336023,-14.7546240064504));
#93254=CARTESIAN_POINT('Ctrl Pts',(17.7207033894106,17.3522587648924,-14.7546233413217));
#93255=CARTESIAN_POINT('Ctrl Pts',(17.7207227775041,17.3522481955641,-14.7546220070071));
#93256=CARTESIAN_POINT('Ctrl Pts',(17.7207325016844,17.3522428945718,-14.7546213377739));
#93257=CARTESIAN_POINT('Ctrl Pts',(17.7207519723628,17.3522322806191,-14.7546199977674));
#93258=CARTESIAN_POINT('Ctrl Pts',(17.720761774882,17.3522269371207,-14.7546193231384));
#93259=CARTESIAN_POINT('Ctrl Pts',(17.7207814225257,17.3522162271022,-14.7546179709444));
#93260=CARTESIAN_POINT('Ctrl Pts',(17.7207912660535,17.3522108614526,-14.7546172934891));
#93261=CARTESIAN_POINT('Ctrl Pts',(17.7208110155964,17.3522000962955,-14.7546159342737));
#93262=CARTESIAN_POINT('Ctrl Pts',(17.7208209197984,17.3521946977775,-14.7546152526384));
#93263=CARTESIAN_POINT('Ctrl Pts',(17.7208408246989,17.3521838483502,-14.7546138827223));
#93264=CARTESIAN_POINT('Ctrl Pts',(17.7208507733133,17.352178425832,-14.7546131980262));
#93265=CARTESIAN_POINT('Ctrl Pts',(17.7238601058545,17.3505382124049,-14.7544060852418));
#93266=CARTESIAN_POINT('Ctrl Pts',(17.7268633780036,17.348910718339,-14.7541991891587));
#93267=CARTESIAN_POINT('Ctrl Pts',(17.7339045057823,17.3451170993749,-14.7537136658549));
#93268=CARTESIAN_POINT('Ctrl Pts',(17.7379454510664,17.3429568176735,-14.7534346722837));
#93269=CARTESIAN_POINT('Ctrl Pts',(17.7503890311355,17.3363563586983,-14.7525745515342));
#93270=CARTESIAN_POINT('Ctrl Pts',(17.7588144426734,17.331959702139,-14.7519907829509));
#93271=CARTESIAN_POINT('Ctrl Pts',(17.8740984783587,17.2727848922271,-14.7439871942518));
#93272=CARTESIAN_POINT('Ctrl Pts',(17.9853878363025,17.2271447679186,-14.7360866505523));
#93273=CARTESIAN_POINT('Ctrl Pts',(18.2037525158422,17.1585945596431,-14.720966304644));
#93274=CARTESIAN_POINT('Ctrl Pts',(18.3099420885646,17.1340529968721,-14.7137743028233));
#93275=CARTESIAN_POINT('Ctrl Pts',(18.4915160222587,17.1066031891036,-14.701977063376));
#93276=CARTESIAN_POINT('Ctrl Pts',(18.5660248641103,17.0993487744956,-14.6972713587155));
#93277=CARTESIAN_POINT('Ctrl Pts',(18.6595270652887,17.0952270135606,-14.691538005017));
#93278=CARTESIAN_POINT('Ctrl Pts',(18.6782957390707,17.0946496936655,-14.690395604011));
#93279=CARTESIAN_POINT('Ctrl Pts',(18.7056173573618,17.0941730104952,-14.6887444653229));
#93280=CARTESIAN_POINT('Ctrl Pts',(18.7141655386271,17.0940756566685,-14.6882295559854));
#93281=CARTESIAN_POINT('Ctrl Pts',(18.72916239922,17.0939957065688,-14.6873290948004));
#93282=CARTESIAN_POINT('Ctrl Pts',(18.7356108021183,17.0939907918172,-14.6869428489901));
#93283=CARTESIAN_POINT('Ctrl Pts',(18.7481384103832,17.0940384833689,-14.686194257091));
#93284=CARTESIAN_POINT('Ctrl Pts',(18.7542175582907,17.0940878126224,-14.6858318122002));
#93285=CARTESIAN_POINT('Ctrl Pts',(18.7687596470708,17.0942684620982,-14.6849667114913));
#93286=CARTESIAN_POINT('Ctrl Pts',(18.7772222205011,17.0944243506482,-14.6844648281934));
#93287=CARTESIAN_POINT('Ctrl Pts',(18.8078153918785,17.0951714647278,-14.6826558841119));
#93288=CARTESIAN_POINT('Ctrl Pts',(18.8299378014056,17.0960590798965,-14.6813580861697));
#93289=CARTESIAN_POINT('Ctrl Pts',(19.0370407923683,17.1076250322666,-14.6692945679292));
#93290=CARTESIAN_POINT('Ctrl Pts',(19.2198767734016,17.1421960510957,-14.6593821587678));
#93291=CARTESIAN_POINT('Ctrl Pts',(19.4722003392099,17.2252498830168,-14.6449018754311));
#93292=CARTESIAN_POINT('Ctrl Pts',(19.5470137817247,17.2546897379911,-14.640484381163));
#93293=CARTESIAN_POINT('Ctrl Pts',(19.6527382783776,17.3034070240085,-14.6338260494439));
#93294=CARTESIAN_POINT('Ctrl Pts',(19.6851158769681,17.3193422019941,-14.6317273177624));
#93295=CARTESIAN_POINT('Ctrl Pts',(19.7236835019477,17.3395643589369,-14.6291357712455));
#93296=CARTESIAN_POINT('Ctrl Pts',(19.7302802445997,17.3430678644241,-14.6286892079536));
#93297=CARTESIAN_POINT('Ctrl Pts',(19.7405218332053,17.3485768190172,-14.6279905470797));
#93298=CARTESIAN_POINT('Ctrl Pts',(19.7441796170762,17.3505582658033,-14.6277399490601));
#93299=CARTESIAN_POINT('Ctrl Pts',(19.7509618393948,17.354258140612,-14.627273255934));
#93300=CARTESIAN_POINT('Ctrl Pts',(19.7540877849913,17.355973686037,-14.6270573446658));
#93301=CARTESIAN_POINT('Ctrl Pts',(19.7611572579809,17.3598767453571,-14.6265672174679));
#93302=CARTESIAN_POINT('Ctrl Pts',(19.7650981188443,17.3620689561403,-14.6262927043333));
#93303=CARTESIAN_POINT('Ctrl Pts',(19.7752541316709,17.3677610813809,-14.6255819716341));
#93304=CARTESIAN_POINT('Ctrl Pts',(19.7814585950792,17.3712798130904,-14.6251445865443));
#93305=CARTESIAN_POINT('Ctrl Pts',(19.8194282038753,17.3930678205638,-14.6224488534005));
#93306=CARTESIAN_POINT('Ctrl Pts',(19.8507303166432,17.4121267910756,-14.6201443732444));
#93307=CARTESIAN_POINT('Ctrl Pts',(20.0248080780698,17.5244124701656,-14.6069248120852));
#93308=CARTESIAN_POINT('Ctrl Pts',(20.1564044248614,17.6338089110355,-14.5954194463102));
#93309=CARTESIAN_POINT('Ctrl Pts',(20.3389498886409,17.8271907158452,-14.5781372887802));
#93310=CARTESIAN_POINT('Ctrl Pts',(20.3996851144032,17.9009276224433,-14.5720752770046));
#93311=CARTESIAN_POINT('Ctrl Pts',(20.4677003530977,17.9959157150026,-14.5648990210767));
#93312=CARTESIAN_POINT('Ctrl Pts',(20.4798919036987,18.0134991660483,-14.5635949282936));
#93313=CARTESIAN_POINT('Ctrl Pts',(20.4968363305516,18.0387465045181,-14.5617560378387));
#93314=CARTESIAN_POINT('Ctrl Pts',(20.5018097355606,18.046260145456,-14.5612129289374));
#93315=CARTESIAN_POINT('Ctrl Pts',(20.5103025631564,18.0592705184964,-14.5602795451815));
#93316=CARTESIAN_POINT('Ctrl Pts',(20.51384478594,18.0647521498893,-14.5598884192364));
#93317=CARTESIAN_POINT('Ctrl Pts',(20.520575666109,18.0752746962347,-14.559141650114));
#93318=CARTESIAN_POINT('Ctrl Pts',(20.5237684741472,18.0803128697931,-14.55878585492));
#93319=CARTESIAN_POINT('Ctrl Pts',(20.5320092863036,18.0934390386526,-14.5578633963749));
#93320=CARTESIAN_POINT('Ctrl Pts',(20.5370240587277,18.1015478180062,-14.5572979643667));
#93321=CARTESIAN_POINT('Ctrl Pts',(20.5539058222054,18.1292620543609,-14.5553801709333));
#93322=CARTESIAN_POINT('Ctrl Pts',(20.565509436491,18.1490266344562,-14.5540374285452));
#93323=CARTESIAN_POINT('Ctrl Pts',(20.663650729255,18.3225868076299,-14.5424505459645));
#93324=CARTESIAN_POINT('Ctrl Pts',(20.7309644217023,18.486452080381,-14.5329671870379));
#93325=CARTESIAN_POINT('Ctrl Pts',(20.7997638421875,18.7400872461869,-14.5186656755487));
#93326=CARTESIAN_POINT('Ctrl Pts',(20.8172426869461,18.8246884344534,-14.513938285898));
#93327=CARTESIAN_POINT('Ctrl Pts',(20.8348593197461,18.9473781500297,-14.5068602610292));
#93328=CARTESIAN_POINT('Ctrl Pts',(20.839214783305,18.9847773591439,-14.5046731125794));
#93329=CARTESIAN_POINT('Ctrl Pts',(20.8432447319754,19.0298016571566,-14.501983519773));
#93330=CARTESIAN_POINT('Ctrl Pts',(20.8438784832334,19.0373366449291,-14.5015315107062));
#93331=CARTESIAN_POINT('Ctrl Pts',(20.844799862241,19.0490419353556,-14.5008261683893));
#93332=CARTESIAN_POINT('Ctrl Pts',(20.8451155358369,19.0532100548362,-14.5005743814444));
#93333=CARTESIAN_POINT('Ctrl Pts',(20.8456774806304,19.0609336157271,-14.5001066198758));
#93334=CARTESIAN_POINT('Ctrl Pts',(20.8459271190536,19.0644887543152,-14.4998908363447));
#93335=CARTESIAN_POINT('Ctrl Pts',(20.8464705010979,19.0725172255188,-14.4994024729696));
#93336=CARTESIAN_POINT('Ctrl Pts',(20.8467590119133,19.0769908452358,-14.4991296050961));
#93337=CARTESIAN_POINT('Ctrl Pts',(20.847566800596,19.0901678888321,-14.4983237548342));
#93338=CARTESIAN_POINT('Ctrl Pts',(20.8480465146547,19.098873519893,-14.497788636437));
#93339=CARTESIAN_POINT('Ctrl Pts',(20.8510777739034,19.1608501102201,-14.4939608922289));
#93340=CARTESIAN_POINT('Ctrl Pts',(20.8516690202901,19.2141933166927,-14.4905712491947));
#93341=CARTESIAN_POINT('Ctrl Pts',(20.849771296706,19.2852779855699,-14.4859755175017));
#93342=CARTESIAN_POINT('Ctrl Pts',(20.8490725191469,19.3030522291724,-14.4848197735307));
#93343=CARTESIAN_POINT('Ctrl Pts',(20.8456417841853,19.3691003570406,-14.4805049749309));
#93344=CARTESIAN_POINT('Ctrl Pts',(20.8414803257243,19.4172842432429,-14.4773175553088));
#93345=CARTESIAN_POINT('Ctrl Pts',(20.8225348262352,19.5738711838925,-14.466898421102));
#93346=CARTESIAN_POINT('Ctrl Pts',(20.8009994148964,19.681287253838,-14.4596657481459));
#93347=CARTESIAN_POINT('Ctrl Pts',(20.7562766792513,19.8395872832691,-14.4490923647354));
#93348=CARTESIAN_POINT('Ctrl Pts',(20.7392311683564,19.8920093410287,-14.4456032762369));
#93349=CARTESIAN_POINT('Ctrl Pts',(20.7082857979193,19.97589297996,-14.4400457747291));
#93350=CARTESIAN_POINT('Ctrl Pts',(20.6956323716152,20.0077837458202,-14.4379389241457));
#93351=CARTESIAN_POINT('Ctrl Pts',(20.6779797130102,20.0493010776704,-14.4352024119854));
#93352=CARTESIAN_POINT('Ctrl Pts',(20.673674356959,20.0592153129718,-14.4345494094366));
#93353=CARTESIAN_POINT('Ctrl Pts',(20.6664971896164,20.0754022180398,-14.4334839121122));
#93354=CARTESIAN_POINT('Ctrl Pts',(20.6636703519265,20.0816945027249,-14.4330698879061));
#93355=CARTESIAN_POINT('Ctrl Pts',(20.6581380617941,20.0938495957112,-14.4322703730626));
#93356=CARTESIAN_POINT('Ctrl Pts',(20.6554364460723,20.0997140567263,-14.4318847560845));
#93357=CARTESIAN_POINT('Ctrl Pts',(20.6491353965626,20.1132288478629,-14.4309963348185));
#93358=CARTESIAN_POINT('Ctrl Pts',(20.6455168633236,20.1208701915526,-14.4304941966003));
#93359=CARTESIAN_POINT('Ctrl Pts',(20.6356595230338,20.1413678076158,-14.4291475832915));
#93360=CARTESIAN_POINT('Ctrl Pts',(20.6293360948846,20.1541830688318,-14.4283060496316));
#93361=CARTESIAN_POINT('Ctrl Pts',(20.5701244976835,20.2711826181164,-14.4206240565047));
#93362=CARTESIAN_POINT('Ctrl Pts',(20.5088231053038,20.370891616978,-14.4141002963679));
#93363=CARTESIAN_POINT('Ctrl Pts',(20.3431651249008,20.5961995976273,-14.3987908013014));
#93364=CARTESIAN_POINT('Ctrl Pts',(20.2319380122963,20.7157791069975,-14.3901882912071));
#93365=CARTESIAN_POINT('Ctrl Pts',(20.0834417584139,20.8424867616726,-14.378979084769));
#93366=CARTESIAN_POINT('Ctrl Pts',(20.0582758625374,20.8629792047038,-14.3770862664228));
#93367=CARTESIAN_POINT('Ctrl Pts',(20.0269361876511,20.8873225735431,-14.3747234574541));
#93368=CARTESIAN_POINT('Ctrl Pts',(20.0211991957322,20.8917318593329,-14.3742906996231));
#93369=CARTESIAN_POINT('Ctrl Pts',(20.0121692051913,20.8985986980074,-14.3736089913711));
#93370=CARTESIAN_POINT('Ctrl Pts',(20.0088914014812,20.9010762693989,-14.3733614248366));
#93371=CARTESIAN_POINT('Ctrl Pts',(20.0027505658338,20.9056898717341,-14.3728973653981));
#93372=CARTESIAN_POINT('Ctrl Pts',(19.999889333394,20.9078282042104,-14.3726810375456));
#93373=CARTESIAN_POINT('Ctrl Pts',(19.9933448682973,20.9126934226707,-14.372186000265));
#93374=CARTESIAN_POINT('Ctrl Pts',(19.9896581970831,20.9154155870131,-14.3719069685211));
#93375=CARTESIAN_POINT('Ctrl Pts',(19.978296550821,20.9237479305096,-14.3710466156867));
#93376=CARTESIAN_POINT('Ctrl Pts',(19.9705927238708,20.9293183079316,-14.3704626511641));
#93377=CARTESIAN_POINT('Ctrl Pts',(19.8655500875889,21.0041988632052,-14.3624950877892));
#93378=CARTESIAN_POINT('Ctrl Pts',(19.7625612688421,21.0651906197424,-14.3546353179602));
#93379=CARTESIAN_POINT('Ctrl Pts',(19.5568295753698,21.164593123943,-14.3395409607983));
#93380=CARTESIAN_POINT('Ctrl Pts',(19.4551412751722,21.2043723536813,-14.3323343131133));
#93381=CARTESIAN_POINT('Ctrl Pts',(19.2789768596638,21.2580300245103,-14.3205014679587));
#93382=CARTESIAN_POINT('Ctrl Pts',(19.205998412301,21.2760790180474,-14.3157751883983));
#93383=CARTESIAN_POINT('Ctrl Pts',(19.1137242387055,21.2937512229167,-14.3100196277815));
#93384=CARTESIAN_POINT('Ctrl Pts',(19.0951943511194,21.2970445418641,-14.30887459241));
#93385=CARTESIAN_POINT('Ctrl Pts',(19.0681789154828,21.3014752246207,-14.3072203719711));
#93386=CARTESIAN_POINT('Ctrl Pts',(19.0597268875907,21.3028088369554,-14.3067049828028));
#93387=CARTESIAN_POINT('Ctrl Pts',(19.0448902189832,21.3050577518684,-14.3058039682094));
#93388=CARTESIAN_POINT('Ctrl Pts',(19.0385090919058,21.3059951815683,-14.3054176461905));
#93389=CARTESIAN_POINT('Ctrl Pts',(19.026107334211,21.3077592218988,-14.3046691139596));
#93390=CARTESIAN_POINT('Ctrl Pts',(19.0200872387001,21.3085890975963,-14.3043068039707));
#93391=CARTESIAN_POINT('Ctrl Pts',(19.0056828708493,21.3105115873742,-14.3034423553043));
#93392=CARTESIAN_POINT('Ctrl Pts',(18.9972954208162,21.311579922869,-14.3029409864763));
#93393=CARTESIAN_POINT('Ctrl Pts',(18.9669802968281,21.3152568281218,-14.3011358535905));
#93394=CARTESIAN_POINT('Ctrl Pts',(18.9450180565557,21.3175725839205,-14.2998413006809));
#93395=CARTESIAN_POINT('Ctrl Pts',(18.7379199827263,21.336138137842,-14.2877478434002));
#93396=CARTESIAN_POINT('Ctrl Pts',(18.5514434170283,21.3282875468118,-14.2778083650023));
#93397=CARTESIAN_POINT('Ctrl Pts',(18.2608025090816,21.2773254224045,-14.2617216768859));
#93398=CARTESIAN_POINT('Ctrl Pts',(18.1548646586907,21.2501695597091,-14.2557003810084));
#93399=CARTESIAN_POINT('Ctrl Pts',(18.040343472846,21.2111671856347,-14.248559775022));
#93400=CARTESIAN_POINT('Ctrl Pts',(18.0292094441632,21.207271125442,-14.2478586791554));
#93401=CARTESIAN_POINT('Ctrl Pts',(18.0134002024229,21.2015903560976,-14.2468526045614));
#93402=CARTESIAN_POINT('Ctrl Pts',(18.0086976288879,21.199881721809,-14.2465519988798));
#93403=CARTESIAN_POINT('Ctrl Pts',(18.0005936629115,21.1969046611281,-14.2460315741936));
#93404=CARTESIAN_POINT('Ctrl Pts',(17.9971893597688,21.1956441138572,-14.2458122242128));
#93405=CARTESIAN_POINT('Ctrl Pts',(17.9905867710304,21.193179973797,-14.2453853522918));
#93406=CARTESIAN_POINT('Ctrl Pts',(17.987388151527,21.1919773913057,-14.2451778966455));
#93407=CARTESIAN_POINT('Ctrl Pts',(17.9787483398747,21.1887051903587,-14.2446157842747));
#93408=CARTESIAN_POINT('Ctrl Pts',(17.9733127973195,21.1866208816299,-14.2442602608719));
#93409=CARTESIAN_POINT('Ctrl Pts',(17.9530677564887,21.1787617999759,-14.24292924112));
#93410=CARTESIAN_POINT('Ctrl Pts',(17.9383152763305,21.1728428725006,-14.2419456234424));
#93411=CARTESIAN_POINT('Ctrl Pts',(17.8094129752262,21.1194321996078,-14.2332390236098));
#93412=CARTESIAN_POINT('Ctrl Pts',(17.6995707159296,21.0621955459608,-14.2250578474201));
#93413=CARTESIAN_POINT('Ctrl Pts',(17.4544611345086,20.9058165199231,-14.2058447694268));
#93414=CARTESIAN_POINT('Ctrl Pts',(17.3246749611485,20.7995359555036,-14.1949287920433));
#93415=CARTESIAN_POINT('Ctrl Pts',(17.1939622374886,20.6637305902117,-14.1833517514888));
#93416=CARTESIAN_POINT('Ctrl Pts',(17.1794267472057,20.6481654502522,-14.1820538228942));
#93417=CARTESIAN_POINT('Ctrl Pts',(17.1590898228379,20.6257182815798,-14.1802220395227));
#93418=CARTESIAN_POINT('Ctrl Pts',(17.1530939482356,20.6190148940125,-14.1796799605968));
#93419=CARTESIAN_POINT('Ctrl Pts',(17.1428229801553,20.6073836313759,-14.1787477914602));
#93420=CARTESIAN_POINT('Ctrl Pts',(17.1385276479695,20.6024738696221,-14.178356855997));
#93421=CARTESIAN_POINT('Ctrl Pts',(17.1303461927102,20.5930344006403,-14.1776100726829));
#93422=CARTESIAN_POINT('Ctrl Pts',(17.1264564025671,20.5885079679131,-14.1772540746334));
#93423=CARTESIAN_POINT('Ctrl Pts',(17.1163900583104,20.5766933557242,-14.1763302732042));
#93424=CARTESIAN_POINT('Ctrl Pts',(17.1102435596605,20.5693796569169,-14.1757637084269));
#93425=CARTESIAN_POINT('Ctrl Pts',(17.089446485294,20.5442904153736,-14.1738378781157));
#93426=CARTESIAN_POINT('Ctrl Pts',(17.0750362878584,20.5263170939052,-14.1724883432209));
#93427=CARTESIAN_POINT('Ctrl Pts',(16.953766337136,20.3698971700147,-14.1609878265011));
#93428=CARTESIAN_POINT('Ctrl Pts',(16.864150154017,20.2189398915557,-14.1515817994359));
#93429=CARTESIAN_POINT('Ctrl Pts',(16.7591127275801,19.9785619014972,-14.1373097817773));
#93430=CARTESIAN_POINT('Ctrl Pts',(16.7291075080056,19.8963719336705,-14.1325252751382));
#93431=CARTESIAN_POINT('Ctrl Pts',(16.6934927506757,19.7762058875582,-14.125370235814));
#93432=CARTESIAN_POINT('Ctrl Pts',(16.6836950214513,19.7395608976502,-14.1231672807582));
#93433=CARTESIAN_POINT('Ctrl Pts',(16.6731275270582,19.6953047300112,-14.1204601680526));
#93434=CARTESIAN_POINT('Ctrl Pts',(16.6714072198997,19.6879249844417,-14.1200072134695));
#93435=CARTESIAN_POINT('Ctrl Pts',(16.6687987127009,19.6764569208378,-14.1193007114558));
#93436=CARTESIAN_POINT('Ctrl Pts',(16.6678829298,19.6723748516669,-14.1190487185104));
#93437=CARTESIAN_POINT('Ctrl Pts',(16.6662094767309,19.6648105900958,-14.1185807699362));
#93438=CARTESIAN_POINT('Ctrl Pts',(16.6654484969531,19.6613291890014,-14.1183650066512));
#93439=CARTESIAN_POINT('Ctrl Pts',(16.6637510234887,19.6534683397513,-14.1178769403347));
#93440=CARTESIAN_POINT('Ctrl Pts',(16.6628196396638,19.6490878570938,-14.117604350828));
#93441=CARTESIAN_POINT('Ctrl Pts',(16.6601202351964,19.6361909880336,-14.1168000668043));
#93442=CARTESIAN_POINT('Ctrl Pts',(16.6583908184045,19.6276667427219,-14.1162662484183));
#93443=CARTESIAN_POINT('Ctrl Pts',(16.6465063451288,19.5671778946155,-14.11246366245));
#93444=CARTESIAN_POINT('Ctrl Pts',(16.6382522854133,19.5148633783206,-14.1090992546497));
#93445=CARTESIAN_POINT('Ctrl Pts',(16.6301911557542,19.4474349068513,-14.1047115460807));
#93446=CARTESIAN_POINT('Ctrl Pts',(16.6285718207931,19.4325519920709,-14.1037398732529));
#93447=CARTESIAN_POINT('Ctrl Pts',(16.6204362485765,19.3496075534794,-14.0983107806219));
#93448=CARTESIAN_POINT('Ctrl Pts',(16.6170625895926,19.281280122789,-14.0937881882882));
#93449=CARTESIAN_POINT('Ctrl Pts',(16.6168557116705,19.0521414080326,-14.0786472548159));
#93450=CARTESIAN_POINT('Ctrl Pts',(16.6350247738266,18.8918491647295,-14.0681492543664));
#93451=CARTESIAN_POINT('Ctrl Pts',(16.6765204048253,18.7119688441873,-14.0567777517569));
#93452=CARTESIAN_POINT('Ctrl Pts',(16.6822553156487,18.6888906229362,-14.0553254722581));
#93453=CARTESIAN_POINT('Ctrl Pts',(16.6908695980434,18.6565626266136,-14.053299773467));
#93454=CARTESIAN_POINT('Ctrl Pts',(16.6934253016897,18.6472291725468,-14.0527159507125));
#93455=CARTESIAN_POINT('Ctrl Pts',(16.6976666649288,18.632146446195,-14.0517740690389));
#93456=CARTESIAN_POINT('Ctrl Pts',(16.6993128687432,18.6263863093291,-14.051414733227));
#93457=CARTESIAN_POINT('Ctrl Pts',(16.7027975173184,18.6143864002933,-14.0506668861545));
#93458=CARTESIAN_POINT('Ctrl Pts',(16.7046403176352,18.6081479501106,-14.0502785213764));
#93459=CARTESIAN_POINT('Ctrl Pts',(16.7090695304346,18.5934041602845,-14.0493616221231));
#93460=CARTESIAN_POINT('Ctrl Pts',(16.7116808336732,18.5849063800131,-14.0488339074799));
#93461=CARTESIAN_POINT('Ctrl Pts',(16.7205471773943,18.5566875633133,-14.0470838258043));
#93462=CARTESIAN_POINT('Ctrl Pts',(16.7270378948414,18.5370414056753,-14.0458691950132));
#93463=CARTESIAN_POINT('Ctrl Pts',(16.7375951451554,18.5065926190859,-14.0439912513117));
#93464=CARTESIAN_POINT('Ctrl Pts',(16.7414631935575,18.4957244434831,-14.0433218631904));
#93465=CARTESIAN_POINT('Ctrl Pts',(16.7454194461219,18.4848895533475,-14.0426552599844));
#93466=CARTESIAN_POINT('Origin',(18.734,19.211,0.));
#93467=CARTESIAN_POINT('',(16.7454194503191,18.4848895418526,-13.2445592875761));
#93468=CARTESIAN_POINT('',(16.7454194857027,18.4848894449486,-13.4647888259555));
#93469=CARTESIAN_POINT('',(16.7454194503191,18.4848895418526,0.));
#93470=CARTESIAN_POINT('',(16.6170008950802,19.2090532671895,-13.5109437209775));
#93471=CARTESIAN_POINT('Ctrl Pts',(16.7454194857027,18.4848894449486,-13.4647888259555));
#93472=CARTESIAN_POINT('Ctrl Pts',(16.729766689791,18.5277573591082,-13.4673502383313));
#93473=CARTESIAN_POINT('Ctrl Pts',(16.7154972638857,18.5711390561076,-13.4699562830825));
#93474=CARTESIAN_POINT('Ctrl Pts',(16.6982006737283,18.6300882848655,-13.4735579023356));
#93475=CARTESIAN_POINT('Ctrl Pts',(16.6939331614507,18.6452574976678,-13.4744899974107));
#93476=CARTESIAN_POINT('Ctrl Pts',(16.688327079247,18.666073447028,-13.4757780725209));
#93477=CARTESIAN_POINT('Ctrl Pts',(16.6868416780844,18.6716805677099,-13.4761259264936));
#93478=CARTESIAN_POINT('Ctrl Pts',(16.6845188929975,18.68059652954,-13.4766805685755));
#93479=CARTESIAN_POINT('Ctrl Pts',(16.6836664223905,18.6839014612219,-13.4768864907921));
#93480=CARTESIAN_POINT('Ctrl Pts',(16.6819231277774,18.6907282368419,-13.4773125581594));
#93481=CARTESIAN_POINT('Ctrl Pts',(16.6810333782027,18.6942503061859,-13.4775327661828));
#93482=CARTESIAN_POINT('Ctrl Pts',(16.6789361643699,18.702643026039,-13.478058406022));
#93483=CARTESIAN_POINT('Ctrl Pts',(16.6777369481559,18.7075156984371,-13.4783643090191));
#93484=CARTESIAN_POINT('Ctrl Pts',(16.6752325955531,18.7178496140955,-13.4790145326324));
#93485=CARTESIAN_POINT('Ctrl Pts',(16.6739318425285,18.7233118684068,-13.4793590913189));
#93486=CARTESIAN_POINT('Ctrl Pts',(16.6704195232459,18.7383259631485,-13.480308434029));
#93487=CARTESIAN_POINT('Ctrl Pts',(16.6682525895442,18.7478879646503,-13.4809155409754));
#93488=CARTESIAN_POINT('Ctrl Pts',(16.633616461448,18.9058077670562,-13.4909794231096));
#93489=CARTESIAN_POINT('Ctrl Pts',(16.6171414693839,19.0572035914288,-13.5011355845678));
#93490=CARTESIAN_POINT('Ctrl Pts',(16.6170009071414,19.2090401949666,-13.5111420663959));
#93491=CARTESIAN_POINT('Ctrl Pts',(16.6170008950802,19.2090532671895,-13.5109437209775));
#93492=CARTESIAN_POINT('Ctrl Pts',(16.6169347298129,19.2810055201563,-13.5152699622426));
#93493=CARTESIAN_POINT('Ctrl Pts',(16.62054107027,19.3530526998715,-13.5195962035077));
#93494=CARTESIAN_POINT('Ctrl Pts',(16.6278222442379,19.4247855494018,-13.5239224447728));
#93495=CARTESIAN_POINT('Ctrl Pts',(16.6350987839402,19.4964727429596,-13.5282459325052));
#93496=CARTESIAN_POINT('Ctrl Pts',(16.6460454699347,19.5678455121798,-13.5325694202375));
#93497=CARTESIAN_POINT('Ctrl Pts',(16.6606126061973,19.6384970353346,-13.5368929079699));
#93498=CARTESIAN_POINT('Ctrl Pts',(16.6751755434729,19.70912819314,-13.5412151494539));
#93499=CARTESIAN_POINT('Ctrl Pts',(16.6933567603002,19.7790380332547,-13.545537390938));
#93500=CARTESIAN_POINT('Ctrl Pts',(16.7150553040206,19.8478291093979,-13.5498596324221));
#93501=CARTESIAN_POINT('Ctrl Pts',(16.7367551488124,19.9166243103389,-13.5541821330731));
#93502=CARTESIAN_POINT('Ctrl Pts',(16.7619725873318,19.9843001434081,-13.5585046337241));
#93503=CARTESIAN_POINT('Ctrl Pts',(16.7905571249898,20.0504753073033,-13.5628271343751));
#93504=CARTESIAN_POINT('Ctrl Pts',(16.8191715095119,20.1167195687348,-13.5671541484134));
#93505=CARTESIAN_POINT('Ctrl Pts',(16.851159810165,20.1814595804034,-13.5714811624517));
#93506=CARTESIAN_POINT('Ctrl Pts',(16.8863242283784,20.2443359777741,-13.57580817649));
#93507=CARTESIAN_POINT('Ctrl Pts',(16.9215100988957,20.3072507333393,-13.580137830254));
#93508=CARTESIAN_POINT('Ctrl Pts',(16.9598756760648,20.3682991960106,-13.5844674840181));
#93509=CARTESIAN_POINT('Ctrl Pts',(17.0011797410095,20.4271508746994,-13.5887971377822));
#93510=CARTESIAN_POINT('Ctrl Pts',(17.0425525940393,20.4861005653946,-13.5931340021826));
#93511=CARTESIAN_POINT('Ctrl Pts',(17.0868733907403,20.5428457872301,-13.597470866583));
#93512=CARTESIAN_POINT('Ctrl Pts',(17.1338612235974,20.5970897865047,-13.6018077309834));
#93513=CARTESIAN_POINT('Ctrl Pts',(17.1504345250049,20.6162224447881,-13.6033374069974));
#93514=CARTESIAN_POINT('Ctrl Pts',(17.167339302115,20.6350442778642,-13.6048670830114));
#93515=CARTESIAN_POINT('Ctrl Pts',(17.1845622179522,20.6535434342032,-13.6063967590254));
#93516=CARTESIAN_POINT('Ctrl Pts',(17.2339699045479,20.7066122947449,-13.6107849679563));
#93517=CARTESIAN_POINT('Ctrl Pts',(17.2862036327226,20.7572434590661,-13.6151731768872));
#93518=CARTESIAN_POINT('Ctrl Pts',(17.3409933109756,20.8051208750698,-13.6195613858181));
#93519=CARTESIAN_POINT('Ctrl Pts',(17.3957016722616,20.8529272330498,-13.6239430819193));
#93520=CARTESIAN_POINT('Ctrl Pts',(17.45295809287,20.8979876412173,-13.6283247780206));
#93521=CARTESIAN_POINT('Ctrl Pts',(17.5124544762692,20.9400215537851,-13.6327064741219));
#93522=CARTESIAN_POINT('Ctrl Pts',(17.5718809466832,20.9820060731604,-13.6370830213815));
#93523=CARTESIAN_POINT('Ctrl Pts',(17.6335417591178,21.0209708847354,-13.6414595686412));
#93524=CARTESIAN_POINT('Ctrl Pts',(17.6970957742218,21.0566756558408,-13.6458361159008));
#93525=CARTESIAN_POINT('Ctrl Pts',(17.760609484293,21.0923577834992,-13.6502098876178));
#93526=CARTESIAN_POINT('Ctrl Pts',(17.8260135952856,21.1247837371303,-13.6545836593348));
#93527=CARTESIAN_POINT('Ctrl Pts',(17.8929392167481,21.1537572568069,-13.6589574310518));
#93528=CARTESIAN_POINT('Ctrl Pts',(17.9598444725194,21.1827219597441,-13.6633298718153));
#93529=CARTESIAN_POINT('Ctrl Pts',(18.0282698771526,21.2082361229382,-13.6677023125789));
#93530=CARTESIAN_POINT('Ctrl Pts',(18.0978247669417,21.2301508296418,-13.6720747533424));
#93531=CARTESIAN_POINT('Ctrl Pts',(18.1673814352569,21.2520660967068,-13.6764473059098));
#93532=CARTESIAN_POINT('Ctrl Pts',(18.2380671853858,21.2703815814966,-13.6808198584771));
#93533=CARTESIAN_POINT('Ctrl Pts',(18.3094759435911,21.2849981498377,-13.6851924110445));
#93534=CARTESIAN_POINT('Ctrl Pts',(18.3809588124992,21.2996298878047,-13.6895695016118));
#93535=CARTESIAN_POINT('Ctrl Pts',(18.4531657140476,21.3105549478119,-13.6939465921792));
#93536=CARTESIAN_POINT('Ctrl Pts',(18.5256809453904,21.3177254618214,-13.6983236827465));
#93537=CARTESIAN_POINT('Ctrl Pts',(18.5982357799925,21.3248998919147,-13.7027031638054));
#93538=CARTESIAN_POINT('Ctrl Pts',(18.6710987974701,21.3283156708867,-13.7070826448644));
#93539=CARTESIAN_POINT('Ctrl Pts',(18.7438524696382,21.3279770732915,-13.7114621259233));
#93540=CARTESIAN_POINT('Ctrl Pts',(18.8167350972017,21.3276378755344,-13.7158493695831));
#93541=CARTESIAN_POINT('Ctrl Pts',(18.8895075103818,21.3235310394329,-13.7202366132428));
#93542=CARTESIAN_POINT('Ctrl Pts',(18.9617560691006,21.3157128481073,-13.7246238569025));
#93543=CARTESIAN_POINT('Ctrl Pts',(19.0108781271737,21.3103972313651,-13.7276067598373));
#93544=CARTESIAN_POINT('Ctrl Pts',(19.0597581560651,21.3033670563132,-13.730589662772));
#93545=CARTESIAN_POINT('Ctrl Pts',(19.1082694567066,21.2946533717911,-13.7335725657068));
#93546=CARTESIAN_POINT('Ctrl Pts',(19.1796354137561,21.2818344939807,-13.7379607746377));
#93547=CARTESIAN_POINT('Ctrl Pts',(19.2504813367646,21.2653198837036,-13.7423489835686));
#93548=CARTESIAN_POINT('Ctrl Pts',(19.3203952805281,21.2451655721633,-13.7467371924995));
#93549=CARTESIAN_POINT('Ctrl Pts',(19.3902054604073,21.2250411729629,-13.7511188886007));
#93550=CARTESIAN_POINT('Ctrl Pts',(19.4590859472337,21.201287928559,-13.755500584702));
#93551=CARTESIAN_POINT('Ctrl Pts',(19.5266340795883,21.1740130452636,-13.7598822808033));
#93552=CARTESIAN_POINT('Ctrl Pts',(19.5941028375116,21.1467702121268,-13.7642588280629));
#93553=CARTESIAN_POINT('Ctrl Pts',(19.660241906012,21.116014140384,-13.7686353753226));
#93554=CARTESIAN_POINT('Ctrl Pts',(19.7246645510875,21.0819015867273,-13.7730119225822));
#93555=CARTESIAN_POINT('Ctrl Pts',(19.7890463402578,21.0478106667563,-13.7773856942992));
#93556=CARTESIAN_POINT('Ctrl Pts',(19.8517134405363,21.0103677135302,-13.7817594660162));
#93557=CARTESIAN_POINT('Ctrl Pts',(19.9123011549783,20.9697766737641,-13.7861332377331));
#93558=CARTESIAN_POINT('Ctrl Pts',(19.9728704323752,20.9291979859878,-13.7905056784967));
#93559=CARTESIAN_POINT('Ctrl Pts',(20.031361179655,20.885473381869,-13.7948781192602));
#93560=CARTESIAN_POINT('Ctrl Pts',(20.087436722545,20.8388507419498,-13.7992505600238));
#93561=CARTESIAN_POINT('Ctrl Pts',(20.1435136992929,20.7922269098846,-13.8036231125911));
#93562=CARTESIAN_POINT('Ctrl Pts',(20.1971749793962,20.7427052048248,-13.8079956651585));
#93563=CARTESIAN_POINT('Ctrl Pts',(20.2481174066912,20.6905734110732,-13.8123682177258));
#93564=CARTESIAN_POINT('Ctrl Pts',(20.2991127039588,20.6383875129796,-13.8167453082932));
#93565=CARTESIAN_POINT('Ctrl Pts',(20.3473831767925,20.5835864635391,-13.8211223988605));
#93566=CARTESIAN_POINT('Ctrl Pts',(20.3926635636817,20.5264938929979,-13.8254994894278));
#93567=CARTESIAN_POINT('Ctrl Pts',(20.4379686798708,20.4693701420848,-13.8298789704868));
#93568=CARTESIAN_POINT('Ctrl Pts',(20.4802801788317,20.409952771581,-13.8342584515457));
#93569=CARTESIAN_POINT('Ctrl Pts',(20.5193756547004,20.3485951703498,-13.8386379326046));
#93570=CARTESIAN_POINT('Ctrl Pts',(20.5585404270376,20.2871288131823,-13.8430251762644));
#93571=CARTESIAN_POINT('Ctrl Pts',(20.5944775548135,20.2237157776927,-13.8474124199241));
#93572=CARTESIAN_POINT('Ctrl Pts',(20.6270104676965,20.1587343347117,-13.8517996635838));
#93573=CARTESIAN_POINT('Ctrl Pts',(20.6491297135927,20.114553215082,-13.8547825665186));
#93574=CARTESIAN_POINT('Ctrl Pts',(20.6696762814796,20.0696475457982,-13.8577654694534));
#93575=CARTESIAN_POINT('Ctrl Pts',(20.6886076987149,20.0241406668741,-13.8607483723882));
#93576=CARTESIAN_POINT('Ctrl Pts',(20.7164580900962,19.9571945754736,-13.8651365813191));
#93577=CARTESIAN_POINT('Ctrl Pts',(20.7409194707721,19.8886853205153,-13.86952479025));
#93578=CARTESIAN_POINT('Ctrl Pts',(20.761815975992,19.8189896113518,-13.8739129991809));
#93579=CARTESIAN_POINT('Ctrl Pts',(20.7826814673334,19.7493973421763,-13.8782946952822));
#93580=CARTESIAN_POINT('Ctrl Pts',(20.7999924489195,19.678622572649,-13.8826763913834));
#93581=CARTESIAN_POINT('Ctrl Pts',(20.8136211113039,19.607061906044,-13.8870580874847));
#93582=CARTESIAN_POINT('Ctrl Pts',(20.8272337589253,19.5355853289173,-13.8914346347443));
#93583=CARTESIAN_POINT('Ctrl Pts',(20.8371725931961,19.4633251607436,-13.895811182004));
#93584=CARTESIAN_POINT('Ctrl Pts',(20.8433600899068,19.3906914330412,-13.9001877292636));
#93585=CARTESIAN_POINT('Ctrl Pts',(20.849543662597,19.3181037685932,-13.9045615009806));
#93586=CARTESIAN_POINT('Ctrl Pts',(20.8519805772149,19.2451434941231,-13.9089352726976));
#93587=CARTESIAN_POINT('Ctrl Pts',(20.8506449171335,19.1722276545358,-13.9133090444145));
#93588=CARTESIAN_POINT('Ctrl Pts',(20.849309663498,19.0993340034833,-13.9176814851781));
#93589=CARTESIAN_POINT('Ctrl Pts',(20.8442041231405,19.0264852424758,-13.9220539259416));
#93590=CARTESIAN_POINT('Ctrl Pts',(20.8353544889709,18.9540986343324,-13.9264263667052));
#93591=CARTESIAN_POINT('Ctrl Pts',(20.8265046285152,18.8817101752555,-13.9307989192725));
#93592=CARTESIAN_POINT('Ctrl Pts',(20.8139105446929,18.8097843710748,-13.9351714718399));
#93593=CARTESIAN_POINT('Ctrl Pts',(20.7976501258783,18.7387319003335,-13.9395440244072));
#93594=CARTESIAN_POINT('Ctrl Pts',(20.7813728313877,18.667605688658,-13.9439211149745));
#93595=CARTESIAN_POINT('Ctrl Pts',(20.7614217126854,18.5973550912948,-13.9482982055419));
#93596=CARTESIAN_POINT('Ctrl Pts',(20.7379253105681,18.5283783261098,-13.9526752961092));
#93597=CARTESIAN_POINT('Ctrl Pts',(20.7144160761935,18.4593638901533,-13.9570547771681));
#93598=CARTESIAN_POINT('Ctrl Pts',(20.6873578824891,18.391625119753,-13.9614342582271));
#93599=CARTESIAN_POINT('Ctrl Pts',(20.656927489488,18.3255403057331,-13.965813739286));
#93600=CARTESIAN_POINT('Ctrl Pts',(20.6264431588197,18.259338356824,-13.9702009829457));
#93601=CARTESIAN_POINT('Ctrl Pts',(20.592574916967,18.1947966461511,-13.9745882266055));
#93602=CARTESIAN_POINT('Ctrl Pts',(20.5555452556645,18.1322683922466,-13.9789754702652));
#93603=CARTESIAN_POINT('Ctrl Pts',(20.5303686541483,18.0897552047994,-13.9819583732));
#93604=CARTESIAN_POINT('Ctrl Pts',(20.5037315602571,18.0481722056908,-13.9849412761348));
#93605=CARTESIAN_POINT('Ctrl Pts',(20.475714693788,18.0076218693017,-13.9879241790697));
#93606=CARTESIAN_POINT('Ctrl Pts',(20.434498513999,17.9479674480279,-13.9923123880006));
#93607=CARTESIAN_POINT('Ctrl Pts',(20.3901335538168,17.8903165376487,-13.9967005969315));
#93608=CARTESIAN_POINT('Ctrl Pts',(20.3428413739373,17.8350209182159,-14.0010888058624));
#93609=CARTESIAN_POINT('Ctrl Pts',(20.2956193834939,17.7798073666505,-14.0054705019636));
#93610=CARTESIAN_POINT('Ctrl Pts',(20.2454791086755,17.7269425302634,-14.0098521980649));
#93611=CARTESIAN_POINT('Ctrl Pts',(20.1926848492424,17.6767485504029,-14.0142338941661));
#93612=CARTESIAN_POINT('Ctrl Pts',(20.1399526272656,17.6266135524633,-14.0186104414258));
#93613=CARTESIAN_POINT('Ctrl Pts',(20.0845729637369,17.5791435071862,-14.0229869886854));
#93614=CARTESIAN_POINT('Ctrl Pts',(20.0268486678901,17.5346255424474,-14.027363535945));
#93615=CARTESIAN_POINT('Ctrl Pts',(19.9691609799527,17.4901358103547,-14.031737307662));
#93616=CARTESIAN_POINT('Ctrl Pts',(19.909131991,17.4485947380415,-14.036111079379));
#93617=CARTESIAN_POINT('Ctrl Pts',(19.8470983416195,17.4102498557868,-14.040484851096));
#93618=CARTESIAN_POINT('Ctrl Pts',(19.7850835692869,17.3719166420085,-14.0448572918595));
#93619=CARTESIAN_POINT('Ctrl Pts',(19.7210657576846,17.3367779408325,-14.0492297326231));
#93620=CARTESIAN_POINT('Ctrl Pts',(19.6554099365357,17.3050375846168,-14.0536021733866));
#93621=CARTESIAN_POINT('Ctrl Pts',(19.5897524365603,17.2732964167967,-14.057974725954));
#93622=CARTESIAN_POINT('Ctrl Pts',(19.5224572790425,17.2449539746122,-14.0623472785213));
#93623=CARTESIAN_POINT('Ctrl Pts',(19.4539119391454,17.2201670587726,-14.0667198310886));
#93624=CARTESIAN_POINT('Ctrl Pts',(19.3852954603089,17.1953544181369,-14.0710969216559));
#93625=CARTESIAN_POINT('Ctrl Pts',(19.3154266631739,17.1741048356878,-14.0754740122233));
#93626=CARTESIAN_POINT('Ctrl Pts',(19.2447099626415,17.1565257767354,-14.0798511027906));
#93627=CARTESIAN_POINT('Ctrl Pts',(19.1739546410942,17.1389371172064,-14.0842305838495));
#93628=CARTESIAN_POINT('Ctrl Pts',(19.1023509680274,17.1250230644095,-14.0886100649085));
#93629=CARTESIAN_POINT('Ctrl Pts',(19.0303127030118,17.114839752778,-14.0929895459674));
#93630=CARTESIAN_POINT('Ctrl Pts',(18.958146750655,17.104638391295,-14.0973767896271));
#93631=CARTESIAN_POINT('Ctrl Pts',(18.8855451489732,17.0981810190707,-14.1017640332868));
#93632=CARTESIAN_POINT('Ctrl Pts',(18.8129253294102,17.0954717462587,-14.1061512769466));
#93633=CARTESIAN_POINT('Ctrl Pts',(18.7635508497362,17.0936297018115,-14.1091341798814));
#93634=CARTESIAN_POINT('Ctrl Pts',(18.7141679744274,17.093519193629,-14.1121170828162));
#93635=CARTESIAN_POINT('Ctrl Pts',(18.6649065603162,17.0951278165748,-14.1150999857511));
#93636=CARTESIAN_POINT('Ctrl Pts',(18.5924370961486,17.0974942943756,-14.119488194682));
#93637=CARTESIAN_POINT('Ctrl Pts',(18.5199478924754,17.1035928606293,-14.1238764036129));
#93638=CARTESIAN_POINT('Ctrl Pts',(18.4478546672521,17.1134276297237,-14.1282646125438));
#93639=CARTESIAN_POINT('Ctrl Pts',(18.3758684403283,17.1232478023901,-14.132646308645));
#93640=CARTESIAN_POINT('Ctrl Pts',(18.3042774991947,17.1367931053665,-14.1370280047463));
#93641=CARTESIAN_POINT('Ctrl Pts',(18.2334957741926,17.1540156733828,-14.1414097008476));
#93642=CARTESIAN_POINT('Ctrl Pts',(18.1627972233503,17.171218003511,-14.1457862481072));
#93643=CARTESIAN_POINT('Ctrl Pts',(18.0929064660602,17.192088901349,-14.1501627953668));
#93644=CARTESIAN_POINT('Ctrl Pts',(18.0242288363214,17.2165291691252,-14.1545393426265));
#93645=CARTESIAN_POINT('Ctrl Pts',(17.9555947609373,17.2409539372388,-14.1589131143435));
#93646=CARTESIAN_POINT('Ctrl Pts',(17.888172739959,17.2689434226001,-14.1632868860604));
#93647=CARTESIAN_POINT('Ctrl Pts',(17.8223531243435,17.300348547195,-14.1676606577774));
#93648=CARTESIAN_POINT('Ctrl Pts',(17.7565535378581,17.331744115105,-14.172033098541));
#93649=CARTESIAN_POINT('Ctrl Pts',(17.6923558237627,17.3665530511359,-14.1764055393045));
#93650=CARTESIAN_POINT('Ctrl Pts',(17.6301289564787,17.4045787536471,-14.1807779800681));
#93651=CARTESIAN_POINT('Ctrl Pts',(17.5679004980471,17.4426054284796,-14.1851505326354));
#93652=CARTESIAN_POINT('Ctrl Pts',(17.5076433970478,17.4838487798649,-14.1895230852027));
#93653=CARTESIAN_POINT('Ctrl Pts',(17.4496992310202,17.5280678757603,-14.1938956377701));
#93654=CARTESIAN_POINT('Ctrl Pts',(17.3916949283512,17.5723328639015,-14.1982727283374));
#93655=CARTESIAN_POINT('Ctrl Pts',(17.3360087376082,17.6195794693658,-14.2026498189047));
#93656=CARTESIAN_POINT('Ctrl Pts',(17.2829499222257,17.6695258121554,-14.2070269094721));
#93657=CARTESIAN_POINT('Ctrl Pts',(17.2298621294548,17.7194994324966,-14.211406390531));
#93658=CARTESIAN_POINT('Ctrl Pts',(17.1794049028391,17.7721753771409,-14.21578587159));
#93659=CARTESIAN_POINT('Ctrl Pts',(17.1318494027618,17.8272361242722,-14.2201653526489));
#93660=CARTESIAN_POINT('Ctrl Pts',(17.0842096108798,17.8823944662081,-14.2245525963086));
#93661=CARTESIAN_POINT('Ctrl Pts',(17.0394821127485,17.9399456706587,-14.2289398399683));
#93662=CARTESIAN_POINT('Ctrl Pts',(16.9978963120797,17.999540968588,-14.2333270836281));
#93663=CARTESIAN_POINT('Ctrl Pts',(16.9696219748233,18.0400600285906,-14.2363099865629));
#93664=CARTESIAN_POINT('Ctrl Pts',(16.9427990411459,18.0815233957323,-14.2392928894977));
#93665=CARTESIAN_POINT('Ctrl Pts',(16.9174873693316,18.1238151663023,-14.2422757924325));
#93666=CARTESIAN_POINT('Ctrl Pts',(16.8789822269094,18.1881511240784,-14.2468135054362));
#93667=CARTESIAN_POINT('Ctrl Pts',(16.8438347836024,18.2546416817585,-14.2513512184399));
#93668=CARTESIAN_POINT('Ctrl Pts',(16.812283422931,18.3229153208065,-14.2558889314436));
#93669=CARTESIAN_POINT('Ctrl Pts',(16.7877996092446,18.3758955734034,-14.259410190666));
#93670=CARTESIAN_POINT('Ctrl Pts',(16.7654805065503,18.4299488289352,-14.2629314498885));
#93671=CARTESIAN_POINT('Ctrl Pts',(16.7454194503191,18.4848895418526,-14.2664527091109));
#93672=CARTESIAN_POINT('',(16.6170000012625,19.2109341693971,-13.288902674305));
#93673=CARTESIAN_POINT('Ctrl Pts',(16.7454194461219,18.4848895533475,-14.0426552599844));
#93674=CARTESIAN_POINT('Ctrl Pts',(16.772186960543,18.4115820298175,-14.0381451053267));
#93675=CARTESIAN_POINT('Ctrl Pts',(16.8029921867809,18.3397980179233,-14.0337655819529));
#93676=CARTESIAN_POINT('Ctrl Pts',(16.8976427044821,18.1490857001761,-14.0220205001263));
#93677=CARTESIAN_POINT('Ctrl Pts',(16.9689849518298,18.0343140293839,-14.0148420577156));
#93678=CARTESIAN_POINT('Ctrl Pts',(17.0971457051432,17.8662887412611,-14.0031497934935));
#93679=CARTESIAN_POINT('Ctrl Pts',(17.1467942049591,17.8080333367713,-13.9988302088228));
#93680=CARTESIAN_POINT('Ctrl Pts',(17.2060220522024,17.7457141580633,-13.9937348316427));
#93681=CARTESIAN_POINT('Ctrl Pts',(17.2126111809091,17.7388738976982,-13.9931687017829));
#93682=CARTESIAN_POINT('Ctrl Pts',(17.2224462449038,17.7288005427014,-13.9923243422884));
#93683=CARTESIAN_POINT('Ctrl Pts',(17.2256571117592,17.7255331655166,-13.9920487855116));
#93684=CARTESIAN_POINT('Ctrl Pts',(17.2313903512507,17.7197367764892,-13.9915568833361));
#93685=CARTESIAN_POINT('Ctrl Pts',(17.2339085440865,17.7172037013116,-13.991340866976));
#93686=CARTESIAN_POINT('Ctrl Pts',(17.2393381903972,17.711769541655,-13.9908751700234));
#93687=CARTESIAN_POINT('Ctrl Pts',(17.2422516423897,17.7088706017064,-13.9906253338696));
#93688=CARTESIAN_POINT('Ctrl Pts',(17.2503213435166,17.7008877267193,-13.9899335183858));
#93689=CARTESIAN_POINT('Ctrl Pts',(17.2554952068252,17.6958217904527,-13.9894901677374));
#93690=CARTESIAN_POINT('Ctrl Pts',(17.284054811362,17.6681435048652,-13.9870445275097));
#93691=CARTESIAN_POINT('Ctrl Pts',(17.307932019281,17.6460472658879,-13.9850059114159));
#93692=CARTESIAN_POINT('Ctrl Pts',(17.4542418809832,17.516779730233,-13.9726000423114));
#93693=CARTESIAN_POINT('Ctrl Pts',(17.5881860853029,17.4234671841384,-13.9616427791892));
#93694=CARTESIAN_POINT('Ctrl Pts',(17.8343782967887,17.2911003264758,-13.9433846914952));
#93695=CARTESIAN_POINT('Ctrl Pts',(17.9416765422598,17.244387351351,-13.9359438477381));
#93696=CARTESIAN_POINT('Ctrl Pts',(18.0658261081519,17.2021603260421,-13.9279367871828));
#93697=CARTESIAN_POINT('Ctrl Pts',(18.0794008269881,17.1976959683585,-13.9270688110954));
#93698=CARTESIAN_POINT('Ctrl Pts',(18.1010776420156,17.1908094724633,-13.9256945024792));
#93699=CARTESIAN_POINT('Ctrl Pts',(18.1091506623598,17.1882978995226,-13.9251852418818));
#93700=CARTESIAN_POINT('Ctrl Pts',(18.1234152322038,17.1839536437119,-13.9242898637858));
#93701=CARTESIAN_POINT('Ctrl Pts',(18.1296004856164,17.1821008113632,-13.92390309016));
#93702=CARTESIAN_POINT('Ctrl Pts',(18.1424111057155,17.1783270889427,-13.9231050215036));
#93703=CARTESIAN_POINT('Ctrl Pts',(18.1490375854781,17.1764102235303,-13.9226938618534));
#93704=CARTESIAN_POINT('Ctrl Pts',(18.1660708893333,17.1715730333901,-13.9216411523522));
#93705=CARTESIAN_POINT('Ctrl Pts',(18.1764910048977,17.1686999354118,-13.9210011438014));
#93706=CARTESIAN_POINT('Ctrl Pts',(18.2200727024244,17.157041730456,-13.9183404806011));
#93707=CARTESIAN_POINT('Ctrl Pts',(18.2534244414615,17.1489832276731,-13.9163433546428));
#93708=CARTESIAN_POINT('Ctrl Pts',(18.3408210818376,17.1301021427088,-13.9111992837305));
#93709=CARTESIAN_POINT('Ctrl Pts',(18.3951196385407,17.1205726991408,-13.9080917276388));
#93710=CARTESIAN_POINT('Ctrl Pts',(18.558087380421,17.0984895566629,-13.8989473222286));
#93711=CARTESIAN_POINT('Ctrl Pts',(18.6674211654396,17.0922235216181,-13.893059202318));
#93712=CARTESIAN_POINT('Ctrl Pts',(18.8224676635182,17.0953550632807,-13.8846160999925));
#93713=CARTESIAN_POINT('Ctrl Pts',(18.8681429011629,17.0977594858628,-13.8821158007853));
#93714=CARTESIAN_POINT('Ctrl Pts',(18.9364164280094,17.1035759246098,-13.8783162827748));
#93715=CARTESIAN_POINT('Ctrl Pts',(18.9590965582257,17.1058776445365,-13.877043720576));
#93716=CARTESIAN_POINT('Ctrl Pts',(18.9827750623048,17.1086677079573,-13.8757003527279));
#93717=CARTESIAN_POINT('Ctrl Pts',(18.983815525844,17.1087910901075,-13.8756412934919));
#93718=CARTESIAN_POINT('Ctrl Pts',(19.0033419620488,17.111121310921,-13.874532356538));
#93719=CARTESIAN_POINT('Ctrl Pts',(19.021797634707,17.1135710773078,-13.8734746599374));
#93720=CARTESIAN_POINT('Ctrl Pts',(19.0731066231257,17.1210716594486,-13.8705016082187));
#93721=CARTESIAN_POINT('Ctrl Pts',(19.1058753321376,17.1266530443555,-13.8685655654256));
#93722=CARTESIAN_POINT('Ctrl Pts',(19.1452810068388,17.1343236408959,-13.8661775442856));
#93723=CARTESIAN_POINT('Ctrl Pts',(19.1520584313266,17.135677395663,-13.8657646728492));
#93724=CARTESIAN_POINT('Ctrl Pts',(19.1631803939236,17.1379556399812,-13.8650834176778));
#93725=CARTESIAN_POINT('Ctrl Pts',(19.1675289266338,17.1388606711713,-13.8648161199363));
#93726=CARTESIAN_POINT('Ctrl Pts',(19.1753590643847,17.1405160322012,-13.8643330723287));
#93727=CARTESIAN_POINT('Ctrl Pts',(19.1788416478259,17.1412614675625,-13.8641176045042));
#93728=CARTESIAN_POINT('Ctrl Pts',(19.1864395999814,17.1429078463782,-13.8636461447825));
#93729=CARTESIAN_POINT('Ctrl Pts',(19.1905541150568,17.1438122758649,-13.8633899597197));
#93730=CARTESIAN_POINT('Ctrl Pts',(19.2021937108581,17.146407271562,-13.8626628083845));
#93731=CARTESIAN_POINT('Ctrl Pts',(19.2097122002091,17.1481266680721,-13.8621902364993));
#93732=CARTESIAN_POINT('Ctrl Pts',(19.2565499218101,17.1591076143776,-13.8592290357217));
#93733=CARTESIAN_POINT('Ctrl Pts',(19.2956040176872,17.1694512696271,-13.8566841535996));
#93734=CARTESIAN_POINT('Ctrl Pts',(19.5036481990321,17.2309736327929,-13.8428030798992));
#93735=CARTESIAN_POINT('Ctrl Pts',(19.6660334920268,17.3020258847687,-13.8308761830411));
#93736=CARTESIAN_POINT('Ctrl Pts',(19.8993933048557,17.4410884904146,-13.8132954712525));
#93737=CARTESIAN_POINT('Ctrl Pts',(19.9777034384407,17.4952102720973,-13.807291482931));
#93738=CARTESIAN_POINT('Ctrl Pts',(20.0629554360456,17.5630442267656,-13.800643043298));
#93739=CARTESIAN_POINT('Ctrl Pts',(20.073707399759,17.5717730849976,-13.7998021978815));
#93740=CARTESIAN_POINT('Ctrl Pts',(20.0907853702842,17.5859179154142,-13.7984626409209));
#93741=CARTESIAN_POINT('Ctrl Pts',(20.097166282787,17.5912666851531,-13.7979612272631));
#93742=CARTESIAN_POINT('Ctrl Pts',(20.1084236618522,17.6008167731039,-13.7970749364925));
#93743=CARTESIAN_POINT('Ctrl Pts',(20.1133128050623,17.6050029222795,-13.7966894451928));
#93744=CARTESIAN_POINT('Ctrl Pts',(20.1234437014717,17.6137575184025,-13.7958894311574));
#93745=CARTESIAN_POINT('Ctrl Pts',(20.1286821981731,17.6183296284381,-13.7954750665526));
#93746=CARTESIAN_POINT('Ctrl Pts',(20.1421935539587,17.6302399925289,-13.7944044513535));
#93747=CARTESIAN_POINT('Ctrl Pts',(20.1504316775105,17.637617466541,-13.793749846204));
#93748=CARTESIAN_POINT('Ctrl Pts',(20.18564352839,17.6696513837465,-13.7909434514846));
#93749=CARTESIAN_POINT('Ctrl Pts',(20.2120351048847,17.6949403193713,-13.7888186075554));
#93750=CARTESIAN_POINT('Ctrl Pts',(20.2801018311239,17.7636310703656,-13.7832657133661));
#93751=CARTESIAN_POINT('Ctrl Pts',(20.3206051550771,17.8081484124568,-13.779885786088));
#93752=CARTESIAN_POINT('Ctrl Pts',(20.4657756217887,17.9820490384535,-13.7673389447173));
#93753=CARTESIAN_POINT('Ctrl Pts',(20.556955443388,18.121874937997,-13.7585778867394));
#93754=CARTESIAN_POINT('Ctrl Pts',(20.6551319224734,18.3199681555161,-13.7461585627983));
#93755=CARTESIAN_POINT('Ctrl Pts',(20.6775267384532,18.3699361882389,-13.7430205534932));
#93756=CARTESIAN_POINT('Ctrl Pts',(20.7012336832368,18.4288506413052,-13.7392523631202));
#93757=CARTESIAN_POINT('Ctrl Pts',(20.7044583868121,18.4370105145514,-13.7387289609956));
#93758=CARTESIAN_POINT('Ctrl Pts',(20.7092581730469,18.4493804407384,-13.7379329190124));
#93759=CARTESIAN_POINT('Ctrl Pts',(20.7108707690888,18.4535759677009,-13.7376624753491));
#93760=CARTESIAN_POINT('Ctrl Pts',(20.713738306732,18.4611080448777,-13.7371760996539));
#93761=CARTESIAN_POINT('Ctrl Pts',(20.7149981924803,18.4644426555173,-13.73696046762));
#93762=CARTESIAN_POINT('Ctrl Pts',(20.7177140092992,18.4716860429504,-13.7364914056217));
#93763=CARTESIAN_POINT('Ctrl Pts',(20.7191667931368,18.4755958930546,-13.7362377976135));
#93764=CARTESIAN_POINT('Ctrl Pts',(20.7232064478981,18.4865669386609,-13.7355250579913));
#93765=CARTESIAN_POINT('Ctrl Pts',(20.725767232167,18.4936375799587,-13.7350644183323));
#93766=CARTESIAN_POINT('Ctrl Pts',(20.740681854981,18.5355142391036,-13.7323292424348));
#93767=CARTESIAN_POINT('Ctrl Pts',(20.7521599996268,18.5706228357228,-13.7300077413549));
#93768=CARTESIAN_POINT('Ctrl Pts',(20.7865881523832,18.6860709763428,-13.7223220446735));
#93769=CARTESIAN_POINT('Ctrl Pts',(20.8057014669072,18.7674689253233,-13.7168251389049));
#93770=CARTESIAN_POINT('Ctrl Pts',(20.8507472032,19.0275946055128,-13.6993878992263));
#93771=CARTESIAN_POINT('Ctrl Pts',(20.8586826193205,19.2086589435697,-13.6875184404006));
#93772=CARTESIAN_POINT('Ctrl Pts',(20.8416464663426,19.4110637362939,-13.6750209748159));
#93773=CARTESIAN_POINT('Ctrl Pts',(20.8393920245303,19.433539009473,-13.6736425388368));
#93774=CARTESIAN_POINT('Ctrl Pts',(20.8356813389835,19.4653902656907,-13.6717016151011));
#93775=CARTESIAN_POINT('Ctrl Pts',(20.8345211680315,19.4747985692403,-13.6711298567217));
#93776=CARTESIAN_POINT('Ctrl Pts',(20.8325293674646,19.49010383894,-13.6702021846301));
#93777=CARTESIAN_POINT('Ctrl Pts',(20.8317359901649,19.4960055713757,-13.6698450682893));
#93778=CARTESIAN_POINT('Ctrl Pts',(20.830019674302,19.5083772612346,-13.6690976714534));
#93779=CARTESIAN_POINT('Ctrl Pts',(20.8290916545913,19.5148464594156,-13.6687075557897));
#93780=CARTESIAN_POINT('Ctrl Pts',(20.8268058318289,19.5302723180431,-13.6677789450173));
#93781=CARTESIAN_POINT('Ctrl Pts',(20.8254204598134,19.5392248116207,-13.6672413282709));
#93782=CARTESIAN_POINT('Ctrl Pts',(20.8205241904645,19.5695749222207,-13.6654229726085));
#93783=CARTESIAN_POINT('Ctrl Pts',(20.8167419583552,19.5909278333102,-13.6641508360488));
#93784=CARTESIAN_POINT('Ctrl Pts',(20.7940865938178,19.708300429984,-13.6571921801672));
#93785=CARTESIAN_POINT('Ctrl Pts',(20.76890064198,19.8029857492757,-13.6517121649714));
#93786=CARTESIAN_POINT('Ctrl Pts',(20.6836228057753,20.0525232618312,-13.6372227301703));
#93787=CARTESIAN_POINT('Ctrl Pts',(20.6117481725394,20.2025852827036,-13.6284820837651));
#93788=CARTESIAN_POINT('Ctrl Pts',(20.5026441817471,20.3750673776048,-13.6168430415648));
#93789=CARTESIAN_POINT('Ctrl Pts',(20.4813024986499,20.4068631482235,-13.6146214641122));
#93790=CARTESIAN_POINT('Ctrl Pts',(20.4549201536874,20.4439538222571,-13.6119159865254));
#93791=CARTESIAN_POINT('Ctrl Pts',(20.45069816667,20.4498255342641,-13.6114842039963));
#93792=CARTESIAN_POINT('Ctrl Pts',(20.44377710014,20.4593476589639,-13.6107780840839));
#93793=CARTESIAN_POINT('Ctrl Pts',(20.4410961780586,20.4630112810115,-13.6105049717883));
#93794=CARTESIAN_POINT('Ctrl Pts',(20.4362870973595,20.4695389824007,-13.6100157285358));
#93795=CARTESIAN_POINT('Ctrl Pts',(20.4341634631601,20.4724063303861,-13.6097999127502));
#93796=CARTESIAN_POINT('Ctrl Pts',(20.4295612152127,20.4785875869001,-13.6093326834355));
#93797=CARTESIAN_POINT('Ctrl Pts',(20.4270801657839,20.4818995540754,-13.609081103897));
#93798=CARTESIAN_POINT('Ctrl Pts',(20.4201536805303,20.49108948057,-13.6083796404286));
#93799=CARTESIAN_POINT('Ctrl Pts',(20.4156872878883,20.4969514667016,-13.6079283228567));
#93800=CARTESIAN_POINT('Ctrl Pts',(20.3901521341403,20.5301049351669,-13.605354306403));
#93801=CARTESIAN_POINT('Ctrl Pts',(20.3684510263718,20.5569001624006,-13.6031907385125));
#93802=CARTESIAN_POINT('Ctrl Pts',(20.2977990840365,20.6399073701967,-13.5962518038293));
#93803=CARTESIAN_POINT('Ctrl Pts',(20.2465309439854,20.6940685972412,-13.5913689263735));
#93804=CARTESIAN_POINT('Ctrl Pts',(20.0516358251991,20.8793242132415,-13.5736345637129));
#93805=CARTESIAN_POINT('Ctrl Pts',(19.8929451092822,20.9932311365298,-13.5607885073879));
#93806=CARTESIAN_POINT('Ctrl Pts',(19.7022563751483,21.0937143545054,-13.5475467500893));
#93807=CARTESIAN_POINT('Ctrl Pts',(19.6834527776957,21.1032666889502,-13.5462609631226));
#93808=CARTESIAN_POINT('Ctrl Pts',(19.6570599207315,21.1161819229198,-13.5444832774506));
#93809=CARTESIAN_POINT('Ctrl Pts',(19.6495893727501,21.1197833507891,-13.5439830780212));
#93810=CARTESIAN_POINT('Ctrl Pts',(19.6366465214609,21.1259294175532,-13.543121546231));
#93811=CARTESIAN_POINT('Ctrl Pts',(19.631184185674,21.1284947079627,-13.542759499694));
#93812=CARTESIAN_POINT('Ctrl Pts',(19.6198392828376,21.133763552057,-13.5420107294257));
#93813=CARTESIAN_POINT('Ctrl Pts',(19.613955127098,21.1364635514253,-13.5416241315505));
#93814=CARTESIAN_POINT('Ctrl Pts',(19.6001265799718,21.1427322780808,-13.5407196468724));
#93815=CARTESIAN_POINT('Ctrl Pts',(19.5921723309973,21.1462790756062,-13.5402025181951));
#93816=CARTESIAN_POINT('Ctrl Pts',(19.5661908523827,21.1576725266623,-13.5385233956705));
#93817=CARTESIAN_POINT('Ctrl Pts',(19.5480758285313,21.1653173040109,-13.537368289663));
#93818=CARTESIAN_POINT('Ctrl Pts',(19.4543620796197,21.2033365518719,-13.5314686907377));
#93819=CARTESIAN_POINT('Ctrl Pts',(19.3771580315603,21.229582747823,-13.5268645310888));
#93820=CARTESIAN_POINT('Ctrl Pts',(19.1363832251023,21.2962135020004,-13.5130215469545));
#93821=CARTESIAN_POINT('Ctrl Pts',(18.9693800175131,21.3215961515659,-13.5041631846135));
#93822=CARTESIAN_POINT('Ctrl Pts',(18.7474453267082,21.3286390134784,-13.4916795887112));
#93823=CARTESIAN_POINT('Ctrl Pts',(18.6937030129506,21.3282980144424,-13.4885974125898));
#93824=CARTESIAN_POINT('Ctrl Pts',(18.6313118133552,21.3255260497222,-13.4848913826419));
#93825=CARTESIAN_POINT('Ctrl Pts',(18.6225893090225,21.3250844189912,-13.4843703526577));
#93826=CARTESIAN_POINT('Ctrl Pts',(18.6093910426849,21.3243342691688,-13.4835772200895));
#93827=CARTESIAN_POINT('Ctrl Pts',(18.6049129953709,21.3240654674834,-13.4833072898137));
#93828=CARTESIAN_POINT('Ctrl Pts',(18.5968788155769,21.3235575694124,-13.4828214612585));
#93829=CARTESIAN_POINT('Ctrl Pts',(18.593322405034,21.3233237245459,-13.4826058600526));
#93830=CARTESIAN_POINT('Ctrl Pts',(18.5855986262203,21.3227962697519,-13.4821364250001));
#93831=CARTESIAN_POINT('Ctrl Pts',(18.5814315863527,21.322499308818,-13.4818824107136));
#93832=CARTESIAN_POINT('Ctrl Pts',(18.5697358180239,21.3216310163151,-13.4811674056511));
#93833=CARTESIAN_POINT('Ctrl Pts',(18.5622093155426,21.321031745093,-13.480704891678));
#93834=CARTESIAN_POINT('Ctrl Pts',(18.5173686190228,21.3172199596104,-13.4779357582697));
#93835=CARTESIAN_POINT('Ctrl Pts',(18.4801442511162,21.3130581660376,-13.4755808336327));
#93836=CARTESIAN_POINT('Ctrl Pts',(18.3583168866353,21.2961545684371,-13.467730711479));
#93837=CARTESIAN_POINT('Ctrl Pts',(18.2743769929017,21.2792727550932,-13.4620969643094));
#93838=CARTESIAN_POINT('Ctrl Pts',(18.020077711642,21.2118809968618,-13.44471710258));
#93839=CARTESIAN_POINT('Ctrl Pts',(17.8548271077964,21.1449827020762,-13.4330520983073));
#93840=CARTESIAN_POINT('Ctrl Pts',(17.6799397817977,21.0470737430313,-13.420717269158));
#93841=CARTESIAN_POINT('Ctrl Pts',(17.6602091605669,21.0356048971113,-13.4193243496196));
#93842=CARTESIAN_POINT('Ctrl Pts',(17.6326734614566,21.0189977872508,-13.4173778654637));
#93843=CARTESIAN_POINT('Ctrl Pts',(17.6247115938295,21.0141237837448,-13.416814735823));
#93844=CARTESIAN_POINT('Ctrl Pts',(17.6112424234108,21.0057554035469,-13.4158614750884));
#93845=CARTESIAN_POINT('Ctrl Pts',(17.6057186088762,21.0022879830647,-13.4154703594317));
#93846=CARTESIAN_POINT('Ctrl Pts',(17.5947619970581,20.9953394866808,-13.4146941845989));
#93847=CARTESIAN_POINT('Ctrl Pts',(17.5893289171412,20.9918589906455,-13.414309109558));
#93848=CARTESIAN_POINT('Ctrl Pts',(17.5784352157938,20.9848099054516,-13.4135365808641));
#93849=CARTESIAN_POINT('Ctrl Pts',(17.5729750064291,20.9812408076113,-13.4131491517415));
#93850=CARTESIAN_POINT('Ctrl Pts',(17.5534356229574,20.9683394837786,-13.4117618703299));
#93851=CARTESIAN_POINT('Ctrl Pts',(17.5394515131731,20.9588639096931,-13.4107673956052));
#93852=CARTESIAN_POINT('Ctrl Pts',(17.4132489974387,20.8711274689274,-13.4017735847869));
#93853=CARTESIAN_POINT('Ctrl Pts',(17.3087449610218,20.7823247702269,-13.394217729598));
#93854=CARTESIAN_POINT('Ctrl Pts',(17.1001166252823,20.5669798550728,-13.3778950017079));
#93855=CARTESIAN_POINT('Ctrl Pts',(17.0006189743921,20.4372259685206,-13.3692254413318));
#93856=CARTESIAN_POINT('Ctrl Pts',(16.9097822585343,20.2852981598106,-13.3588208783816));
#93857=CARTESIAN_POINT('Ctrl Pts',(16.9026838643018,20.2731525746587,-13.3579872729009));
#93858=CARTESIAN_POINT('Ctrl Pts',(16.8929614775417,20.2561300444947,-13.3568151139102));
#93859=CARTESIAN_POINT('Ctrl Pts',(16.8902346034894,20.2513118821481,-13.3564829157797));
#93860=CARTESIAN_POINT('Ctrl Pts',(16.8858822859146,20.2435508304247,-13.3559470450458));
#93861=CARTESIAN_POINT('Ctrl Pts',(16.8842448771525,20.2406146306563,-13.3557441357005));
#93862=CARTESIAN_POINT('Ctrl Pts',(16.8808341614646,20.2344641426313,-13.3553187051586));
#93863=CARTESIAN_POINT('Ctrl Pts',(16.8790622197217,20.2312491396409,-13.3550960960329));
#93864=CARTESIAN_POINT('Ctrl Pts',(16.8747876279606,20.2234453939803,-13.354555239141));
#93865=CARTESIAN_POINT('Ctrl Pts',(16.8722936017513,20.2188519759941,-13.3542364477892));
#93866=CARTESIAN_POINT('Ctrl Pts',(16.863585958373,20.2026719080558,-13.3531121280602));
#93867=CARTESIAN_POINT('Ctrl Pts',(16.8574634406875,20.1910369288681,-13.3523011333792));
#93868=CARTESIAN_POINT('Ctrl Pts',(16.8216449256196,20.1214025742036,-13.3474359490934));
#93869=CARTESIAN_POINT('Ctrl Pts',(16.7945337876491,20.0621192387778,-13.3432478442596));
#93870=CARTESIAN_POINT('Ctrl Pts',(16.7016675229783,19.831470838242,-13.3270234145345));
#93871=CARTESIAN_POINT('Ctrl Pts',(16.6555424809737,19.6530311175561,-13.3147001371237));
#93872=CARTESIAN_POINT('Ctrl Pts',(16.6297590820114,19.4445830695436,-13.301396301187));
#93873=CARTESIAN_POINT('Ctrl Pts',(16.6270006060779,19.4182306438173,-13.2997318591792));
#93874=CARTESIAN_POINT('Ctrl Pts',(16.6216845007598,19.356222630682,-13.2958565775225));
#93875=CARTESIAN_POINT('Ctrl Pts',(16.6195337089458,19.3205396234777,-13.2936584446058));
#93876=CARTESIAN_POINT('Ctrl Pts',(16.617898152872,19.2736622878227,-13.2908108231166));
#93877=CARTESIAN_POINT('Ctrl Pts',(16.6175971716277,19.2625040315736,-13.2901359642465));
#93878=CARTESIAN_POINT('Ctrl Pts',(16.6172522422965,19.2444074776532,-13.28904615179));
#93879=CARTESIAN_POINT('Ctrl Pts',(16.617154128961,19.237470537487,-13.2886295088657));
#93880=CARTESIAN_POINT('Ctrl Pts',(16.6170502015178,19.2262073902167,-13.2879548009108));
#93881=CARTESIAN_POINT('Ctrl Pts',(16.6170235456931,19.2218814682278,-13.2876960853544));
#93882=CARTESIAN_POINT('Ctrl Pts',(16.617003429377,19.2153852082466,-13.2873081997628));
#93883=CARTESIAN_POINT('Ctrl Pts',(16.6170000462453,19.2132149325987,-13.28717872004));
#93884=CARTESIAN_POINT('Ctrl Pts',(16.6170000004709,19.2110446506181,-13.2870493445712));
#93885=CARTESIAN_POINT('Ctrl Pts',(16.6170000013281,19.2109250126717,-13.2890562789747));
#93886=CARTESIAN_POINT('Ctrl Pts',(16.6170027225446,19.1341011600434,-13.2844612169082));
#93887=CARTESIAN_POINT('Ctrl Pts',(16.6211915380442,19.0573628289812,-13.2798661548417));
#93888=CARTESIAN_POINT('Ctrl Pts',(16.6295128869012,18.9811674722736,-13.2752710927752));
#93889=CARTESIAN_POINT('Ctrl Pts',(16.6378461991752,18.9048625712073,-13.2706694244908));
#93890=CARTESIAN_POINT('Ctrl Pts',(16.6503238258347,18.8291026016853,-13.2660677562064));
#93891=CARTESIAN_POINT('Ctrl Pts',(16.666841073,18.7543349471174,-13.261466087922));
#93892=CARTESIAN_POINT('Ctrl Pts',(16.6833972601622,18.679391025148,-13.2568535710412));
#93893=CARTESIAN_POINT('Ctrl Pts',(16.7040119873824,18.6054444839208,-13.2522410541604));
#93894=CARTESIAN_POINT('Ctrl Pts',(16.7285306582113,18.5329279395626,-13.2476285372796));
#93895=CARTESIAN_POINT('Ctrl Pts',(16.7339690428732,18.5168433456905,-13.2466054540451));
#93896=CARTESIAN_POINT('Ctrl Pts',(16.7395993072442,18.5008290221139,-13.2455823708106));
#93897=CARTESIAN_POINT('Ctrl Pts',(16.7454194503191,18.4848895418526,-13.2445592875761));
#93898=CARTESIAN_POINT('Origin',(18.734,19.211,0.));
#93899=CARTESIAN_POINT('',(16.7437496504382,18.4842640742323,-12.4443820746265));
#93900=CARTESIAN_POINT('',(16.7454195353148,18.4848893090773,-12.6679318638109));
#93901=CARTESIAN_POINT('',(16.7454194503191,18.4848895418526,0.));
#93902=CARTESIAN_POINT('Ctrl Pts',(16.7454195353148,18.4848893090773,-12.6679318638109));
#93903=CARTESIAN_POINT('Ctrl Pts',(16.7052039069762,18.5950268044879,-12.6745735300496));
#93904=CARTESIAN_POINT('Ctrl Pts',(16.6741842952664,18.7083782324412,-12.6809438201612));
#93905=CARTESIAN_POINT('Ctrl Pts',(16.6289120083485,18.9517192629599,-12.6943852175721));
#93906=CARTESIAN_POINT('Ctrl Pts',(16.6169601910973,19.0815565992033,-12.7014276223083));
#93907=CARTESIAN_POINT('Ctrl Pts',(16.6170011043132,19.2149245295939,-12.7092186109573));
#93908=CARTESIAN_POINT('Ctrl Pts',(16.6170097091036,19.2181996006972,-12.7094102823505));
#93909=CARTESIAN_POINT('Ctrl Pts',(16.617103391712,19.2371333371875,-12.7105204617434));
#93910=CARTESIAN_POINT('Ctrl Pts',(16.6173546002336,19.2527901998201,-12.7114467850276));
#93911=CARTESIAN_POINT('Ctrl Pts',(16.6179364422518,19.2742257229631,-12.7127280872513));
#93912=CARTESIAN_POINT('Ctrl Pts',(16.6181171315258,19.2800083877722,-12.7130750497816));
#93913=CARTESIAN_POINT('Ctrl Pts',(16.618441995659,19.2891982068463,-12.7136286204981));
#93914=CARTESIAN_POINT('Ctrl Pts',(16.6185707051684,19.2926059279293,-12.7138343687611));
#93915=CARTESIAN_POINT('Ctrl Pts',(16.6188536043165,19.2996449963843,-12.7142603779025));
#93916=CARTESIAN_POINT('Ctrl Pts',(16.6190089118102,19.3032762518521,-12.7144807030064));
#93917=CARTESIAN_POINT('Ctrl Pts',(16.6194013908054,19.311930724983,-12.7150071183992));
#93918=CARTESIAN_POINT('Ctrl Pts',(16.619647110743,19.3169535169137,-12.7153136835633));
#93919=CARTESIAN_POINT('Ctrl Pts',(16.6205368812465,19.3339037197371,-12.7163516706919));
#93920=CARTESIAN_POINT('Ctrl Pts',(16.6212639692446,19.3458262879094,-12.7170875202413));
#93921=CARTESIAN_POINT('Ctrl Pts',(16.6311148216221,19.4875998170897,-12.725900906759));
#93922=CARTESIAN_POINT('Ctrl Pts',(16.652094711903,19.6163356545092,-12.7345186157036));
#93923=CARTESIAN_POINT('Ctrl Pts',(16.7254974566956,19.899444657587,-12.7538452517802));
#93924=CARTESIAN_POINT('Ctrl Pts',(16.7841817064134,20.0513962791147,-12.7644510068483));
#93925=CARTESIAN_POINT('Ctrl Pts',(16.8706981570032,20.2161655755375,-12.7759141072705));
#93926=CARTESIAN_POINT('Ctrl Pts',(16.8820773058399,20.2369795314881,-12.7773627487528));
#93927=CARTESIAN_POINT('Ctrl Pts',(16.8985833620852,20.2660015239528,-12.7793842660749));
#93928=CARTESIAN_POINT('Ctrl Pts',(16.9034200610182,20.2743717798231,-12.7799674882416));
#93929=CARTESIAN_POINT('Ctrl Pts',(16.9113457913493,20.2878734848133,-12.7809086614212));
#93930=CARTESIAN_POINT('Ctrl Pts',(16.914399521296,20.2930253997259,-12.7812678855963));
#93931=CARTESIAN_POINT('Ctrl Pts',(16.9208163214209,20.3037471249721,-12.7820157029795));
#93932=CARTESIAN_POINT('Ctrl Pts',(16.9241832932101,20.3093145363157,-12.7824041488162));
#93933=CARTESIAN_POINT('Ctrl Pts',(16.9322154696904,20.3224588056794,-12.783321601295));
#93934=CARTESIAN_POINT('Ctrl Pts',(16.9369029054475,20.3300219867452,-12.7838497853492));
#93935=CARTESIAN_POINT('Ctrl Pts',(16.9526722167393,20.355111133069,-12.7856030608958));
#93936=CARTESIAN_POINT('Ctrl Pts',(16.9639641003298,20.3725041606249,-12.786820376726));
#93937=CARTESIAN_POINT('Ctrl Pts',(17.0256054181123,20.4644639285047,-12.7932712650584));
#93938=CARTESIAN_POINT('Ctrl Pts',(17.0804171160334,20.5359340336159,-12.7983318959407));
#93939=CARTESIAN_POINT('Ctrl Pts',(17.2287601945877,20.7057586991185,-12.8107686852582));
#93940=CARTESIAN_POINT('Ctrl Pts',(17.3274918566426,20.7990122929935,-12.8179808560139));
#93941=CARTESIAN_POINT('Ctrl Pts',(17.49397403342,20.9284717959191,-12.8296567230741));
#93942=CARTESIAN_POINT('Ctrl Pts',(17.5559174155828,20.9715375976412,-12.8339174608333));
#93943=CARTESIAN_POINT('Ctrl Pts',(17.6280873322142,21.0161970053271,-12.8389474680712));
#93944=CARTESIAN_POINT('Ctrl Pts',(17.6361903782605,21.0211362058263,-12.8395131308456));
#93945=CARTESIAN_POINT('Ctrl Pts',(17.6482524128825,21.0283778221811,-12.8403569256539));
#93946=CARTESIAN_POINT('Ctrl Pts',(17.6521862350008,21.0307222173841,-12.8406323900183));
#93947=CARTESIAN_POINT('Ctrl Pts',(17.6592016978509,21.0348723548971,-12.8411241911849));
#93948=CARTESIAN_POINT('Ctrl Pts',(17.6622803319866,21.0366830804448,-12.8413401994724));
#93949=CARTESIAN_POINT('Ctrl Pts',(17.6689124245777,21.0405612472733,-12.8418059520832));
#93950=CARTESIAN_POINT('Ctrl Pts',(17.6724672751306,21.0426261010944,-12.8420558523538));
#93951=CARTESIAN_POINT('Ctrl Pts',(17.6823041924359,21.0483016710118,-12.8427480218648));
#93952=CARTESIAN_POINT('Ctrl Pts',(17.6885987479381,21.0518904694853,-12.8431916646886));
#93953=CARTESIAN_POINT('Ctrl Pts',(17.7233138396346,21.0714475812456,-12.8456418709247));
#93954=CARTESIAN_POINT('Ctrl Pts',(17.7520802240921,21.0867891673616,-12.8476849176515));
#93955=CARTESIAN_POINT('Ctrl Pts',(17.9264327534546,21.1746647794746,-12.8600922840244));
#93956=CARTESIAN_POINT('Ctrl Pts',(18.0796263352478,21.2308859544734,-12.8710454969299));
#93957=CARTESIAN_POINT('Ctrl Pts',(18.3512830812101,21.2963913895576,-12.8892984033384));
#93958=CARTESIAN_POINT('Ctrl Pts',(18.4669061863381,21.3143302605256,-12.8967379696179));
#93959=CARTESIAN_POINT('Ctrl Pts',(18.5976891509857,21.3236553269854,-12.9047438411114));
#93960=CARTESIAN_POINT('Ctrl Pts',(18.6119522492214,21.3245272745922,-12.905611801654));
#93961=CARTESIAN_POINT('Ctrl Pts',(18.6346668396305,21.3256851777068,-12.9069860904373));
#93962=CARTESIAN_POINT('Ctrl Pts',(18.6431129130332,21.3260650151293,-12.9074953466142));
#93963=CARTESIAN_POINT('Ctrl Pts',(18.6580129416594,21.3266456830078,-12.9083907196266));
#93964=CARTESIAN_POINT('Ctrl Pts',(18.6644659223258,21.3268676004277,-12.9087774925651));
#93965=CARTESIAN_POINT('Ctrl Pts',(18.6778148984399,21.3272655357924,-12.9095755623785));
#93966=CARTESIAN_POINT('Ctrl Pts',(18.6847109487929,21.3274373779497,-12.90998672386));
#93967=CARTESIAN_POINT('Ctrl Pts',(18.7024143993206,21.3277919547547,-12.9110394433812));
#93968=CARTESIAN_POINT('Ctrl Pts',(18.7132226663786,21.3279256337554,-12.9116794600636));
#93969=CARTESIAN_POINT('Ctrl Pts',(18.7583375612461,21.3281380695703,-12.9143402016399));
#93970=CARTESIAN_POINT('Ctrl Pts',(18.7926436572675,21.3274656955864,-12.9163373960773));
#93971=CARTESIAN_POINT('Ctrl Pts',(18.8819742401333,21.3235409984975,-12.9214816830752));
#93972=CARTESIAN_POINT('Ctrl Pts',(18.9369157781641,21.3189733581146,-12.9245893824405));
#93973=CARTESIAN_POINT('Ctrl Pts',(19.1001554904761,21.2989598321755,-12.9337340379255));
#93974=CARTESIAN_POINT('Ctrl Pts',(19.2075002130258,21.2772634235775,-12.9396222654781));
#93975=CARTESIAN_POINT('Ctrl Pts',(19.3568792873577,21.2348134725387,-12.9480771111795));
#93976=CARTESIAN_POINT('Ctrl Pts',(19.4006488841573,21.2208205398169,-12.9505891240598));
#93977=CARTESIAN_POINT('Ctrl Pts',(19.4649304433797,21.1979390318556,-12.9543731565326));
#93978=CARTESIAN_POINT('Ctrl Pts',(19.48581374606,21.1901316459796,-12.955617730027));
#93979=CARTESIAN_POINT('Ctrl Pts',(19.5544213984807,21.1632395748825,-12.9597687632216));
#93980=CARTESIAN_POINT('Ctrl Pts',(19.6015704635986,21.1427482232981,-12.9627220878745));
#93981=CARTESIAN_POINT('Ctrl Pts',(19.6550282824944,21.1171631493982,-12.9662396426317));
#93982=CARTESIAN_POINT('Ctrl Pts',(19.6621144097553,21.1137229665191,-12.9667094201342));
#93983=CARTESIAN_POINT('Ctrl Pts',(19.6733817542589,21.1081749640014,-12.9674622573819));
#93984=CARTESIAN_POINT('Ctrl Pts',(19.6775755405013,21.10609264224,-12.9677437720412));
#93985=CARTESIAN_POINT('Ctrl Pts',(19.6849752315678,21.102387855306,-12.9682428555774));
#93986=CARTESIAN_POINT('Ctrl Pts',(19.6881839569367,21.1007711201164,-12.9684600645359));
#93987=CARTESIAN_POINT('Ctrl Pts',(19.694959044111,21.0973357975639,-12.9689203898002));
#93988=CARTESIAN_POINT('Ctrl Pts',(19.6985243123295,21.0955152893888,-12.9691636209902));
#93989=CARTESIAN_POINT('Ctrl Pts',(19.7080948748259,21.0905940660458,-12.9698191778722));
#93990=CARTESIAN_POINT('Ctrl Pts',(19.714090460338,21.0874747173837,-12.970232651474));
#93991=CARTESIAN_POINT('Ctrl Pts',(19.7432955114369,21.0721019314086,-12.9722600090599));
#93992=CARTESIAN_POINT('Ctrl Pts',(19.7662895574433,21.0594469025525,-12.9738973382631));
#93993=CARTESIAN_POINT('Ctrl Pts',(19.8314788515691,21.0219735606818,-12.9786454989434));
#93994=CARTESIAN_POINT('Ctrl Pts',(19.873055014891,20.996115712638,-12.9818039056192));
#93995=CARTESIAN_POINT('Ctrl Pts',(19.9939452209303,20.9149858227036,-12.9913043555429));
#93996=CARTESIAN_POINT('Ctrl Pts',(20.0704124407586,20.8556979152358,-12.9977331918203));
#93997=CARTESIAN_POINT('Ctrl Pts',(20.2478329620457,20.6975679354631,-13.0133686048274));
#93998=CARTESIAN_POINT('Ctrl Pts',(20.3434829207567,20.5934444083241,-13.0224360965622));
#93999=CARTESIAN_POINT('Ctrl Pts',(20.436643474715,20.4691328175676,-13.0319214066967));
#94000=CARTESIAN_POINT('Ctrl Pts',(20.445092924387,20.4576170255684,-13.032788958786));
#94001=CARTESIAN_POINT('Ctrl Pts',(20.4583563850384,20.4391512538863,-13.0341627251219));
#94002=CARTESIAN_POINT('Ctrl Pts',(20.4632463132491,20.4322565809021,-13.0346718638424));
#94003=CARTESIAN_POINT('Ctrl Pts',(20.4717983248134,20.4200441130374,-13.0355671002427));
#94004=CARTESIAN_POINT('Ctrl Pts',(20.4754775950576,20.414738539858,-13.0359538533955));
#94005=CARTESIAN_POINT('Ctrl Pts',(20.4830379611024,20.403729141521,-13.0367519493366));
#94006=CARTESIAN_POINT('Ctrl Pts',(20.4869155667619,20.3980230039669,-13.0371631564015));
#94007=CARTESIAN_POINT('Ctrl Pts',(20.4967985977,20.3833254713842,-13.0382161312676));
#94008=CARTESIAN_POINT('Ctrl Pts',(20.5027632050298,20.3743067686587,-13.0388563562433));
#94009=CARTESIAN_POINT('Ctrl Pts',(20.5273801315396,20.3364580204881,-13.0415191231348));
#94010=CARTESIAN_POINT('Ctrl Pts',(20.5453993509157,20.3072210729232,-13.0435180888477));
#94011=CARTESIAN_POINT('Ctrl Pts',(20.5904982511446,20.2298953114509,-13.0486679704026));
#94012=CARTESIAN_POINT('Ctrl Pts',(20.6164236518648,20.1811624887711,-13.0517793805904));
#94013=CARTESIAN_POINT('Ctrl Pts',(20.6879861440396,20.0329468982281,-13.0609305093062));
#94014=CARTESIAN_POINT('Ctrl Pts',(20.7278477889549,19.9308822305411,-13.0668215209849));
#94015=CARTESIAN_POINT('Ctrl Pts',(20.7744321528768,19.7774945257218,-13.0755495348637));
#94016=CARTESIAN_POINT('Ctrl Pts',(20.7874609051876,19.7282788220588,-13.078333815612));
#94017=CARTESIAN_POINT('Ctrl Pts',(20.802178873281,19.6632971740539,-13.0820406762741));
#94018=CARTESIAN_POINT('Ctrl Pts',(20.8054834256903,19.6479130178728,-13.0829205093056));
#94019=CARTESIAN_POINT('Ctrl Pts',(20.8191178887894,19.5808034153836,-13.0867736962881));
#94020=CARTESIAN_POINT('Ctrl Pts',(20.827683232228,19.5287431522477,-13.0898016468224));
#94021=CARTESIAN_POINT('Ctrl Pts',(20.8353850230393,19.4677986381042,-13.0934472438762));
#94022=CARTESIAN_POINT('Ctrl Pts',(20.8364216868069,19.4591684922929,-13.0939658298833));
#94023=CARTESIAN_POINT('Ctrl Pts',(20.8379117366798,19.4460839204166,-13.0947559640095));
#94024=CARTESIAN_POINT('Ctrl Pts',(20.8384042009665,19.4416339165982,-13.0950253643043));
#94025=CARTESIAN_POINT('Ctrl Pts',(20.8392632774401,19.4336392414121,-13.0955106296755));
#94026=CARTESIAN_POINT('Ctrl Pts',(20.8396350588344,19.4300951799123,-13.0957262006997));
#94027=CARTESIAN_POINT('Ctrl Pts',(20.8404239568601,19.4223873794548,-13.0961960282573));
#94028=CARTESIAN_POINT('Ctrl Pts',(20.8408376718472,19.4182233915687,-13.0964504677323));
#94029=CARTESIAN_POINT('Ctrl Pts',(20.8419662927639,19.4065111164214,-13.0971678461313));
#94030=CARTESIAN_POINT('Ctrl Pts',(20.8426529878326,19.3989602643751,-13.0976323242002));
#94031=CARTESIAN_POINT('Ctrl Pts',(20.8465378407345,19.3535387381931,-13.1004376346023));
#94032=CARTESIAN_POINT('Ctrl Pts',(20.8487560505634,19.3155937455552,-13.1028282215272));
#94033=CARTESIAN_POINT('Ctrl Pts',(20.8527120529054,19.1899309861176,-13.1108564233111));
#94034=CARTESIAN_POINT('Ctrl Pts',(20.8500194568677,19.1021680664631,-13.1166390251248));
#94035=CARTESIAN_POINT('Ctrl Pts',(20.8257290893626,18.8411604580203,-13.1339593777633));
#94036=CARTESIAN_POINT('Ctrl Pts',(20.7881616451049,18.6701165934674,-13.1454065260778));
#94037=CARTESIAN_POINT('Ctrl Pts',(20.7223354003542,18.4838525800512,-13.1575671972136));
#94038=CARTESIAN_POINT('Ctrl Pts',(20.7142945415091,18.4622312576192,-13.1589753569944));
#94039=CARTESIAN_POINT('Ctrl Pts',(20.7024239027215,18.4318416702177,-13.1609503877165));
#94040=CARTESIAN_POINT('Ctrl Pts',(20.6988858334063,18.4229619107927,-13.1615269784075));
#94041=CARTESIAN_POINT('Ctrl Pts',(20.693040799752,18.4085763125025,-13.1624603359689));
#94042=CARTESIAN_POINT('Ctrl Pts',(20.6907705052105,18.4030558061212,-13.1628183350449));
#94043=CARTESIAN_POINT('Ctrl Pts',(20.6859705826036,18.3915231006353,-13.1635658736304));
#94044=CARTESIAN_POINT('Ctrl Pts',(20.68343645292,18.3855128338747,-13.1639552557864));
#94045=CARTESIAN_POINT('Ctrl Pts',(20.6773439865215,18.3712476839298,-13.1648790189078));
#94046=CARTESIAN_POINT('Ctrl Pts',(20.6737607526023,18.3630035207892,-13.1654125457858));
#94047=CARTESIAN_POINT('Ctrl Pts',(20.6615229545414,18.3353307588443,-13.1672024723544));
#94048=CARTESIAN_POINT('Ctrl Pts',(20.6526279692529,18.3160094277984,-13.1684506363171));
#94049=CARTESIAN_POINT('Ctrl Pts',(20.576743556568,18.1575091963893,-13.1786846154419));
#94050=CARTESIAN_POINT('Ctrl Pts',(20.4949970992559,18.0259078674962,-13.1871019308589));
#94051=CARTESIAN_POINT('Ctrl Pts',(20.3152304177142,17.7967489626181,-13.2029186321855));
#94052=CARTESIAN_POINT('Ctrl Pts',(20.2205943327123,17.6975858008316,-13.2103042190342));
#94053=CARTESIAN_POINT('Ctrl Pts',(20.1052749072516,17.5980718968109,-13.2192364117658));
#94054=CARTESIAN_POINT('Ctrl Pts',(20.0933629586772,17.5880199471401,-13.2201585175607));
#94055=CARTESIAN_POINT('Ctrl Pts',(20.0768874423479,17.5744256318437,-13.2214348710614));
#94056=CARTESIAN_POINT('Ctrl Pts',(20.0724184242064,17.570768776883,-13.2217811820341));
#94057=CARTESIAN_POINT('Ctrl Pts',(20.0652882038302,17.5649828880212,-13.2223339698506));
#94058=CARTESIAN_POINT('Ctrl Pts',(20.0626366872115,17.5628418863469,-13.2225395911249));
#94059=CARTESIAN_POINT('Ctrl Pts',(20.0571456049062,17.5584299019976,-13.2229655592243));
#94060=CARTESIAN_POINT('Ctrl Pts',(20.0543053626281,17.5561598357449,-13.2231859712692));
#94061=CARTESIAN_POINT('Ctrl Pts',(20.0475167446075,17.5507626282338,-13.2237129598209));
#94062=CARTESIAN_POINT('Ctrl Pts',(20.043563041487,17.5476422489008,-13.2240200139323));
#94063=CARTESIAN_POINT('Ctrl Pts',(20.0301588921483,17.5371407109705,-13.2250613581153));
#94064=CARTESIAN_POINT('Ctrl Pts',(20.0206570807284,17.5298259059479,-13.2258001140365));
#94065=CARTESIAN_POINT('Ctrl Pts',(19.9093813361156,17.4456580927729,-13.2344533314345));
#94066=CARTESIAN_POINT('Ctrl Pts',(19.8009353596003,17.3780800536971,-13.2428867790967));
#94067=CARTESIAN_POINT('Ctrl Pts',(19.5396983782028,17.246366908696,-13.2622205408024));
#94068=CARTESIAN_POINT('Ctrl Pts',(19.384101406228,17.1895349610642,-13.2730158708654));
#94069=CARTESIAN_POINT('Ctrl Pts',(19.2004915747925,17.1459014922146,-13.2846391282991));
#94070=CARTESIAN_POINT('Ctrl Pts',(19.1774349445044,17.1408280851586,-13.2860807526524));
#94071=CARTESIAN_POINT('Ctrl Pts',(19.1448415465023,17.1342257445272,-13.2880942056105));
#94072=CARTESIAN_POINT('Ctrl Pts',(19.1353724653406,17.1323749175442,-13.2886762707289));
#94073=CARTESIAN_POINT('Ctrl Pts',(19.1200089926158,17.129480871443,-13.2896160792048));
#94074=CARTESIAN_POINT('Ctrl Pts',(19.1141223285347,17.1283978196924,-13.2899750885476));
#94075=CARTESIAN_POINT('Ctrl Pts',(19.1018246015711,17.1261891141695,-13.2907228505603));
#94076=CARTESIAN_POINT('Ctrl Pts',(19.0954127732787,17.1250680317975,-13.2911114541395));
#94077=CARTESIAN_POINT('Ctrl Pts',(19.0802087078043,17.1224818703207,-13.2920299803864));
#94078=CARTESIAN_POINT('Ctrl Pts',(19.0714121427314,17.1210427045038,-13.2925590751139));
#94079=CARTESIAN_POINT('Ctrl Pts',(19.0426191470949,17.1165185402009,-13.2942834805689));
#94080=CARTESIAN_POINT('Ctrl Pts',(19.0225871647994,17.113664582481,-13.2954714796688));
#94081=CARTESIAN_POINT('Ctrl Pts',(18.9749213752585,17.1075695041379,-13.2982724952258));
#94082=CARTESIAN_POINT('Ctrl Pts',(18.9472582218675,17.1045850382485,-13.2998775526848));
#94083=CARTESIAN_POINT('Ctrl Pts',(18.7508359254928,17.0873032062144,-13.3111481900545));
#94084=CARTESIAN_POINT('Ctrl Pts',(18.5809622467596,17.0927569562635,-13.3201753502847));
#94085=CARTESIAN_POINT('Ctrl Pts',(18.3107907901892,17.1341299011228,-13.3351122077079));
#94086=CARTESIAN_POINT('Ctrl Pts',(18.2093464381105,17.1574108875477,-13.3408765536017));
#94087=CARTESIAN_POINT('Ctrl Pts',(18.1007796311637,17.1908973247029,-13.3476075900357));
#94088=CARTESIAN_POINT('Ctrl Pts',(18.0915420544373,17.1938161624729,-13.3481849022349));
#94089=CARTESIAN_POINT('Ctrl Pts',(18.0779311500703,17.1982198353205,-13.3490427707239));
#94090=CARTESIAN_POINT('Ctrl Pts',(18.0735419752895,17.1996557918038,-13.3493205285213));
#94091=CARTESIAN_POINT('Ctrl Pts',(18.0657629029168,17.2022289909374,-13.3498148489441));
#94092=CARTESIAN_POINT('Ctrl Pts',(18.0623711510381,17.2033604721463,-13.3500310700607));
#94093=CARTESIAN_POINT('Ctrl Pts',(18.0551094864893,17.205803409574,-13.3504954971452));
#94094=CARTESIAN_POINT('Ctrl Pts',(18.0512405577055,17.2071174588076,-13.3507438496981));
#94095=CARTESIAN_POINT('Ctrl Pts',(18.0406289265565,17.2107559094706,-13.3514274834749));
#94096=CARTESIAN_POINT('Ctrl Pts',(18.0338942007325,17.2131031724135,-13.3518640841223));
#94097=CARTESIAN_POINT('Ctrl Pts',(17.9984774581856,17.2256480806605,-13.3541740085612));
#94098=CARTESIAN_POINT('Ctrl Pts',(17.9700075820052,17.2364289034281,-13.3560790349566));
#94099=CARTESIAN_POINT('Ctrl Pts',(17.7914208948333,17.3084954257281,-13.3682924678814));
#94100=CARTESIAN_POINT('Ctrl Pts',(17.6485332974991,17.3862423988859,-13.3792084614568));
#94101=CARTESIAN_POINT('Ctrl Pts',(17.4180928270384,17.5483562544187,-13.3976307189773));
#94102=CARTESIAN_POINT('Ctrl Pts',(17.3262603589321,17.6253539589863,-13.405258330257));
#94103=CARTESIAN_POINT('Ctrl Pts',(17.2302711969332,17.7207867640229,-13.4135235169064));
#94104=CARTESIAN_POINT('Ctrl Pts',(17.2192537711696,17.7319869219712,-13.4144773235938));
#94105=CARTESIAN_POINT('Ctrl Pts',(17.2027731932283,17.7491181832114,-13.4159122515394));
#94106=CARTESIAN_POINT('Ctrl Pts',(17.1972177505116,17.7549593753963,-13.416397389438));
#94107=CARTESIAN_POINT('Ctrl Pts',(17.1873222617206,17.7654835745059,-13.4172641789679));
#94108=CARTESIAN_POINT('Ctrl Pts',(17.1829698046096,17.7701547283509,-13.4176463632809));
#94109=CARTESIAN_POINT('Ctrl Pts',(17.1737790452115,17.7801083605335,-13.4184554225023));
#94110=CARTESIAN_POINT('Ctrl Pts',(17.168946279506,17.7853958594475,-13.4188820586169));
#94111=CARTESIAN_POINT('Ctrl Pts',(17.1591628934814,17.7962095095405,-13.4197482692234));
#94112=CARTESIAN_POINT('Ctrl Pts',(17.1542142974444,17.8017373629848,-13.4201877554741));
#94113=CARTESIAN_POINT('Ctrl Pts',(17.1324256418596,17.8263354810243,-13.4221289502548));
#94114=CARTESIAN_POINT('Ctrl Pts',(17.1159006354143,17.8456829001378,-13.4236175525859));
#94115=CARTESIAN_POINT('Ctrl Pts',(17.0457285954405,17.930904173027,-13.4300186729676));
#94116=CARTESIAN_POINT('Ctrl Pts',(16.9957224712622,17.9996787795795,-13.4347858967342));
#94117=CARTESIAN_POINT('Ctrl Pts',(16.9128101383288,18.1294624461232,-13.4432735431789));
#94118=CARTESIAN_POINT('Ctrl Pts',(16.8785074211341,18.1894307972629,-13.4470186741641));
#94119=CARTESIAN_POINT('Ctrl Pts',(16.8085769124412,18.3268692270204,-13.4553932840246));
#94120=CARTESIAN_POINT('Ctrl Pts',(16.7745951535261,18.4049867853306,-13.4600145404506));
#94121=CARTESIAN_POINT('Ctrl Pts',(16.7454194857027,18.4848894449486,-13.4647888259555));
#94122=CARTESIAN_POINT('',(16.6170008459317,19.2091074688849,-12.4890563034237));
#94123=CARTESIAN_POINT('Ctrl Pts',(16.7454194503191,18.4848895418526,-13.2445592875761));
#94124=CARTESIAN_POINT('Ctrl Pts',(16.771739242225,18.4128081860915,-13.2399327109632));
#94125=CARTESIAN_POINT('Ctrl Pts',(16.8019456372607,18.3422595341822,-13.2353061343503));
#94126=CARTESIAN_POINT('Ctrl Pts',(16.8358258585856,18.2736505833652,-13.2306795577375));
#94127=CARTESIAN_POINT('Ctrl Pts',(16.8465556085575,18.251922363793,-13.2292143367814));
#94128=CARTESIAN_POINT('Ctrl Pts',(16.8576534980229,18.23038848217,-13.2277491158253));
#94129=CARTESIAN_POINT('Ctrl Pts',(16.869111861991,18.209061262994,-13.2262838948692));
#94130=CARTESIAN_POINT('Ctrl Pts',(16.9034286623953,18.145188102246,-13.2218956859383));
#94131=CARTESIAN_POINT('Ctrl Pts',(16.9410977666971,18.0829553476818,-13.2175074770074));
#94132=CARTESIAN_POINT('Ctrl Pts',(16.9819381659419,18.0227372640544,-13.2131192680765));
#94133=CARTESIAN_POINT('Ctrl Pts',(17.0227179512629,17.9626085540473,-13.2087375719752));
#94134=CARTESIAN_POINT('Ctrl Pts',(17.0666594195119,17.9044889751322,-13.2043558758739));
#94135=CARTESIAN_POINT('Ctrl Pts',(17.1135357879725,17.8487280970606,-13.1999741797727));
#94136=CARTESIAN_POINT('Ctrl Pts',(17.1603570729695,17.7930327424584,-13.195597632513));
#94137=CARTESIAN_POINT('Ctrl Pts',(17.2101060983657,17.7396909501816,-13.1912210852534));
#94138=CARTESIAN_POINT('Ctrl Pts',(17.2625139124407,17.6890217826396,-13.1868445379937));
#94139=CARTESIAN_POINT('Ctrl Pts',(17.3148884902417,17.6383847487473,-13.1824707662767));
#94140=CARTESIAN_POINT('Ctrl Pts',(17.3699181652077,17.5904173110759,-13.1780969945597));
#94141=CARTESIAN_POINT('Ctrl Pts',(17.4272959551564,17.5454029481326,-13.1737232228428));
#94142=CARTESIAN_POINT('Ctrl Pts',(17.484656284851,17.500402283211,-13.1693507820792));
#94143=CARTESIAN_POINT('Ctrl Pts',(17.5443629316542,17.4583532065242,-13.1649783413156));
#94144=CARTESIAN_POINT('Ctrl Pts',(17.606075834685,17.4194989318177,-13.1606059005521));
#94145=CARTESIAN_POINT('Ctrl Pts',(17.6677903157216,17.380643663603,-13.1562333479847));
#94146=CARTESIAN_POINT('Ctrl Pts',(17.7315107455623,17.3449836148749,-13.1518607954174));
#94147=CARTESIAN_POINT('Ctrl Pts',(17.7968695201159,17.3127177597438,-13.14748824285));
#94148=CARTESIAN_POINT('Ctrl Pts',(17.862296126471,17.2804184178912,-13.1431111522827));
#94149=CARTESIAN_POINT('Ctrl Pts',(17.929364038908,17.2515205167786,-13.1387340617153));
#94150=CARTESIAN_POINT('Ctrl Pts',(17.9976833250416,17.2261758883523,-13.134356971148));
#94151=CARTESIAN_POINT('Ctrl Pts',(18.0660399228729,17.2008174182837,-13.1299774900891));
#94152=CARTESIAN_POINT('Ctrl Pts',(18.1356487944388,17.179016228838,-13.1255980090301));
#94153=CARTESIAN_POINT('Ctrl Pts',(18.2061050046754,17.1608741809559,-13.1212185279712));
#94154=CARTESIAN_POINT('Ctrl Pts',(18.2766860980717,17.1426999764157,-13.1168312843114));
#94155=CARTESIAN_POINT('Ctrl Pts',(18.3481170562262,17.1281979613854,-13.1124440406517));
#94156=CARTESIAN_POINT('Ctrl Pts',(18.4199835016944,17.1174187049957,-13.108056796992));
#94157=CARTESIAN_POINT('Ctrl Pts',(18.4688457595774,17.1100898493375,-13.1050738940572));
#94158=CARTESIAN_POINT('Ctrl Pts',(18.5179091821644,17.1044808253816,-13.1020909911225));
#94159=CARTESIAN_POINT('Ctrl Pts',(18.567043338876,17.1005937658104,-13.0991080881877));
#94160=CARTESIAN_POINT('Ctrl Pts',(18.6393255921075,17.0948754337364,-13.0947198792568));
#94161=CARTESIAN_POINT('Ctrl Pts',(18.7120430618564,17.0928637794812,-13.0903316703259));
#94162=CARTESIAN_POINT('Ctrl Pts',(18.7847830739805,17.0946091855716,-13.085943461395));
#94163=CARTESIAN_POINT('Ctrl Pts',(18.8574151278661,17.0963520011899,-13.0815617652938));
#94164=CARTESIAN_POINT('Ctrl Pts',(18.9300691794581,17.1018407963575,-13.0771800691925));
#94165=CARTESIAN_POINT('Ctrl Pts',(19.0023285427329,17.1110740981752,-13.0727983730912));
#94166=CARTESIAN_POINT('Ctrl Pts',(19.0745029955053,17.1202965501284,-13.0684218258316));
#94167=CARTESIAN_POINT('Ctrl Pts',(19.1462832051704,17.1332547070803,-13.0640452785719));
#94168=CARTESIAN_POINT('Ctrl Pts',(19.2172553122695,17.1498951256272,-13.0596687313123));
#94169=CARTESIAN_POINT('Ctrl Pts',(19.2881824098898,17.1665249910625,-13.0552949595953));
#94170=CARTESIAN_POINT('Ctrl Pts',(19.3583019532985,17.1868323748369,-13.0509211878784));
#94171=CARTESIAN_POINT('Ctrl Pts',(19.4272094182998,17.2107125950553,-13.0465474161614));
#94172=CARTESIAN_POINT('Ctrl Pts',(19.4960959145281,17.2345855484424,-13.0421749753978));
#94173=CARTESIAN_POINT('Ctrl Pts',(19.5637706090995,17.2620290219354,-13.0378025346343));
#94174=CARTESIAN_POINT('Ctrl Pts',(19.6298449292381,17.2928887251365,-13.0334300938707));
#94175=CARTESIAN_POINT('Ctrl Pts',(19.6959209389044,17.3237492174237,-13.0290575413034));
#94176=CARTESIAN_POINT('Ctrl Pts',(19.7603960566788,17.3580259069127,-13.024684988736));
#94177=CARTESIAN_POINT('Ctrl Pts',(19.8229039997004,17.3955173976497,-13.0203124361687));
#94178=CARTESIAN_POINT('Ctrl Pts',(19.885476815823,17.43304779847,-13.0159353456014));
#94179=CARTESIAN_POINT('Ctrl Pts',(19.9460779664252,17.473799413322,-13.011558255034));
#94180=CARTESIAN_POINT('Ctrl Pts',(20.0043687218637,17.5175265545305,-13.0071811644667));
#94181=CARTESIAN_POINT('Ctrl Pts',(20.0626913120471,17.5612775767537,-13.0028016834078));
#94182=CARTESIAN_POINT('Ctrl Pts',(20.1187006241998,17.608007051543,-12.9984222023488));
#94183=CARTESIAN_POINT('Ctrl Pts',(20.1720918257207,17.6574296279874,-12.9940427212899));
#94184=CARTESIAN_POINT('Ctrl Pts',(20.2255776627878,17.7069398056168,-12.9896554776302));
#94185=CARTESIAN_POINT('Ctrl Pts',(20.2764357852884,17.759152271547,-12.9852682339705));
#94186=CARTESIAN_POINT('Ctrl Pts',(20.3243993779349,17.813745972035,-12.9808809903107));
#94187=CARTESIAN_POINT('Ctrl Pts',(20.3570099991736,17.8508644277303,-12.9778980873759));
#94188=CARTESIAN_POINT('Ctrl Pts',(20.3882834007588,17.8890829433879,-12.9749151844411));
#94189=CARTESIAN_POINT('Ctrl Pts',(20.4181471898432,17.9282930019123,-12.9719322815063));
#94190=CARTESIAN_POINT('Ctrl Pts',(20.4620804149045,17.9859757132704,-12.9675440725754));
#94191=CARTESIAN_POINT('Ctrl Pts',(20.5031324849612,18.0460307272458,-12.9631558636445));
#94192=CARTESIAN_POINT('Ctrl Pts',(20.541037663595,18.1081383212981,-12.9587676547136));
#94193=CARTESIAN_POINT('Ctrl Pts',(20.5788865846589,18.1701537373831,-12.9543859586124));
#94194=CARTESIAN_POINT('Ctrl Pts',(20.6135976366773,18.23421527774,-12.9500042625111));
#94195=CARTESIAN_POINT('Ctrl Pts',(20.6449465138837,18.2999717781125,-12.9456225664098));
#94196=CARTESIAN_POINT('Ctrl Pts',(20.6762585536647,18.3656510093639,-12.9412460191502));
#94197=CARTESIAN_POINT('Ctrl Pts',(20.7042160604133,18.4330208108149,-12.9368694718905));
#94198=CARTESIAN_POINT('Ctrl Pts',(20.728639957299,18.5017042642547,-12.9324929246309));
#94199=CARTESIAN_POINT('Ctrl Pts',(20.7530483649042,18.5703441596466,-12.9281191529139));
#94200=CARTESIAN_POINT('Ctrl Pts',(20.7739274477879,18.640295600672,-12.923745381197));
#94201=CARTESIAN_POINT('Ctrl Pts',(20.7911462655828,18.7111617841753,-12.91937160948));
#94202=CARTESIAN_POINT('Ctrl Pts',(20.8083598436336,18.782006402861,-12.9149991687164));
#94203=CARTESIAN_POINT('Ctrl Pts',(20.8219152540693,18.853764742938,-12.9106267279529));
#94204=CARTESIAN_POINT('Ctrl Pts',(20.8317319036235,18.9260265617289,-12.9062542871893));
#94205=CARTESIAN_POINT('Ctrl Pts',(20.8415488041905,18.9982902282625,-12.901881734622));
#94206=CARTESIAN_POINT('Ctrl Pts',(20.847626691118,19.0710569208137,-12.8975091820546));
#94207=CARTESIAN_POINT('Ctrl Pts',(20.8499366445659,19.143909641652,-12.8931366294873));
#94208=CARTESIAN_POINT('Ctrl Pts',(20.8522489953706,19.2168379717919,-12.88875953892));
#94209=CARTESIAN_POINT('Ctrl Pts',(20.8507855897922,19.2898520253122,-12.8843824483526));
#94210=CARTESIAN_POINT('Ctrl Pts',(20.8455696643533,19.3625339981092,-12.8800053577853));
#94211=CARTESIAN_POINT('Ctrl Pts',(20.8403508903039,19.4352556652291,-12.8756258767264));
#94212=CARTESIAN_POINT('Ctrl Pts',(20.8313755754734,19.5076444114925,-12.8712463956674));
#94213=CARTESIAN_POINT('Ctrl Pts',(20.818718654715,19.5792894658868,-12.8668669146085));
#94214=CARTESIAN_POINT('Ctrl Pts',(20.8060392996495,19.6510615106591,-12.8624796709487));
#94215=CARTESIAN_POINT('Ctrl Pts',(20.7896654157131,19.72208676073,-12.858092427289));
#94216=CARTESIAN_POINT('Ctrl Pts',(20.7697225362412,19.7919670863653,-12.8537051836293));
#94217=CARTESIAN_POINT('Ctrl Pts',(20.7561632998915,19.8394789741454,-12.8507222806945));
#94218=CARTESIAN_POINT('Ctrl Pts',(20.7409552755656,19.8864619134098,-12.8477393777596));
#94219=CARTESIAN_POINT('Ctrl Pts',(20.7241505240926,19.9327962949848,-12.8447564748248));
#94220=CARTESIAN_POINT('Ctrl Pts',(20.6994287137936,20.0009597422968,-12.8403682658939));
#94221=CARTESIAN_POINT('Ctrl Pts',(20.6711526578598,20.0679846766149,-12.835980056963));
#94222=CARTESIAN_POINT('Ctrl Pts',(20.6394473542676,20.1334745959182,-12.8315918480321));
#94223=CARTESIAN_POINT('Ctrl Pts',(20.6077891066028,20.1988673173228,-12.8272101519309));
#94224=CARTESIAN_POINT('Ctrl Pts',(20.5727119232316,20.2627291156992,-12.8228284558296));
#94225=CARTESIAN_POINT('Ctrl Pts',(20.5343896652635,20.3246813068434,-12.8184467597283));
#94226=CARTESIAN_POINT('Ctrl Pts',(20.4961124389983,20.3865606992326,-12.8140702124687));
#94227=CARTESIAN_POINT('Ctrl Pts',(20.4545979656272,20.4465345337929,-12.8096936652091));
#94228=CARTESIAN_POINT('Ctrl Pts',(20.4100662428249,20.5042482165705,-12.8053171179494));
#94229=CARTESIAN_POINT('Ctrl Pts',(20.3655627613939,20.5619252981693,-12.8009433462325));
#94230=CARTESIAN_POINT('Ctrl Pts',(20.3180461211089,20.617344690981,-12.7965695745155));
#94231=CARTESIAN_POINT('Ctrl Pts',(20.2677790950909,20.6701815128564,-12.7921958027985));
#94232=CARTESIAN_POINT('Ctrl Pts',(20.2175273654978,20.7230022563095,-12.787823362035));
#94233=CARTESIAN_POINT('Ctrl Pts',(20.1645272440668,20.7732416397748,-12.7834509212714));
#94234=CARTESIAN_POINT('Ctrl Pts',(20.1090800563606,20.8206098404891,-12.7790784805079));
#94235=CARTESIAN_POINT('Ctrl Pts',(20.0536314508637,20.8679792524136,-12.7747059279405));
#94236=CARTESIAN_POINT('Ctrl Pts',(19.9957360229244,20.9124770240216,-12.7703333753732));
#94237=CARTESIAN_POINT('Ctrl Pts',(19.9357287478821,20.9538531253418,-12.7659608228058));
#94238=CARTESIAN_POINT('Ctrl Pts',(19.8756591950264,20.9952721683406,-12.7615837322385));
#94239=CARTESIAN_POINT('Ctrl Pts',(19.8134738170563,21.0335627981877,-12.7572066416712));
#94240=CARTESIAN_POINT('Ctrl Pts',(19.7495364985934,21.068518403684,-12.7528295511039));
#94241=CARTESIAN_POINT('Ctrl Pts',(19.6855642615878,21.1034930997338,-12.7484500700449));
#94242=CARTESIAN_POINT('Ctrl Pts',(19.6198386140603,21.135128935727,-12.744070588986));
#94243=CARTESIAN_POINT('Ctrl Pts',(19.5527455102414,21.163266577458,-12.7396911079271));
#94244=CARTESIAN_POINT('Ctrl Pts',(19.4855334843463,21.1914540929701,-12.7353038642673));
#94245=CARTESIAN_POINT('Ctrl Pts',(19.4169496162067,21.2161308685659,-12.7309166206076));
#94246=CARTESIAN_POINT('Ctrl Pts',(19.3473966187371,21.2371869578402,-12.7265293769479));
#94247=CARTESIAN_POINT('Ctrl Pts',(19.3001072825686,21.2515030695869,-12.7235464740131));
#94248=CARTESIAN_POINT('Ctrl Pts',(19.2523702507341,21.2641465017728,-12.7205635710783));
#94249=CARTESIAN_POINT('Ctrl Pts',(19.2043142751595,21.2750962871391,-12.7175806681434));
#94250=CARTESIAN_POINT('Ctrl Pts',(19.1336181560408,21.2912047381968,-12.7131924592126));
#94251=CARTESIAN_POINT('Ctrl Pts',(19.0619555004259,21.3037083756574,-12.7088042502817));
#94252=CARTESIAN_POINT('Ctrl Pts',(18.9897273628005,21.3124976840137,-12.7044160413508));
#94253=CARTESIAN_POINT('Ctrl Pts',(18.9176064237069,21.3212739475792,-12.7000343452495));
#94254=CARTESIAN_POINT('Ctrl Pts',(18.8449221435536,21.3263467676749,-12.6956526491482));
#94255=CARTESIAN_POINT('Ctrl Pts',(18.7720870435491,21.3276573594027,-12.691270953047));
#94256=CARTESIAN_POINT('Ctrl Pts',(18.6993375305835,21.3289664110809,-12.6868944057873));
#94257=CARTESIAN_POINT('Ctrl Pts',(18.6264380297318,21.3265220079374,-12.6825178585277));
#94258=CARTESIAN_POINT('Ctrl Pts',(18.5538057789622,21.3203171982195,-12.6781413112681));
#94259=CARTESIAN_POINT('Ctrl Pts',(18.4812195905104,21.3141163235017,-12.6737675395511));
#94260=CARTESIAN_POINT('Ctrl Pts',(18.4089007953028,21.3041598149104,-12.6693937678341));
#94261=CARTESIAN_POINT('Ctrl Pts',(18.33726480192,21.2904927705103,-12.6650199961171));
#94262=CARTESIAN_POINT('Ctrl Pts',(18.2656506076105,21.2768298850376,-12.6606475553536));
#94263=CARTESIAN_POINT('Ctrl Pts',(18.1947192761672,21.2594587957696,-12.65627511459));
#94264=CARTESIAN_POINT('Ctrl Pts',(18.1248776044805,21.2384759942541,-12.6519026738265));
#94265=CARTESIAN_POINT('Ctrl Pts',(18.0550341469344,21.217492656206,-12.6475301212591));
#94266=CARTESIAN_POINT('Ctrl Pts',(17.9862808658672,21.1928975632636,-12.6431575686918));
#94267=CARTESIAN_POINT('Ctrl Pts',(17.9190093127144,21.1648370401949,-12.6387850161244));
#94268=CARTESIAN_POINT('Ctrl Pts',(17.8516679426063,21.136747394857,-12.6344079255571));
#94269=CARTESIAN_POINT('Ctrl Pts',(17.7858118168723,21.1051853247306,-12.6300308349898));
#94270=CARTESIAN_POINT('Ctrl Pts',(17.7218116266776,21.0703449644729,-12.6256537444225));
#94271=CARTESIAN_POINT('Ctrl Pts',(17.6577764836036,21.0354855766014,-12.6212742633635));
#94272=CARTESIAN_POINT('Ctrl Pts',(17.5955997055918,20.9973445863421,-12.6168947823046));
#94273=CARTESIAN_POINT('Ctrl Pts',(17.5356241771986,20.9561602755406,-12.6125153012456));
#94274=CARTESIAN_POINT('Ctrl Pts',(17.4755423425838,20.9149029658247,-12.6081280575859));
#94275=CARTESIAN_POINT('Ctrl Pts',(17.4176699324641,20.8705918569496,-12.6037408139262));
#94276=CARTESIAN_POINT('Ctrl Pts',(17.3623173752294,20.8235060548421,-12.5993535702665));
#94277=CARTESIAN_POINT('Ctrl Pts',(17.3246829700695,20.791492246586,-12.5963706673317));
#94278=CARTESIAN_POINT('Ctrl Pts',(17.2882126945401,20.7581966074029,-12.5933877643968));
#94279=CARTESIAN_POINT('Ctrl Pts',(17.2529938697633,20.7237160481073,-12.590404861462));
#94280=CARTESIAN_POINT('Ctrl Pts',(17.2019441492121,20.6737364440846,-12.5860811407752));
#94281=CARTESIAN_POINT('Ctrl Pts',(17.1533139178897,20.6210584681426,-12.5817574200883));
#94282=CARTESIAN_POINT('Ctrl Pts',(17.1074080252022,20.5659492785796,-12.5774336994015));
#94283=CARTESIAN_POINT('Ctrl Pts',(17.0615630887849,20.5109132659108,-12.5731157199794));
#94284=CARTESIAN_POINT('Ctrl Pts',(17.0184356374497,20.453452815078,-12.5687977405574));
#94285=CARTESIAN_POINT('Ctrl Pts',(16.9782947055965,20.3938727400712,-12.5644797611354));
#94286=CARTESIAN_POINT('Ctrl Pts',(16.9381929308677,20.3343507849011,-12.5601659938641));
#94287=CARTESIAN_POINT('Ctrl Pts',(16.9010721765565,20.2727137148021,-12.5558522265928));
#94288=CARTESIAN_POINT('Ctrl Pts',(16.867160867601,20.2092988799672,-12.5515384593216));
#94289=CARTESIAN_POINT('Ctrl Pts',(16.8332706976893,20.1459235755725,-12.5472273810917));
#94290=CARTESIAN_POINT('Ctrl Pts',(16.8025862384803,20.0807731423996,-12.5429163028619));
#94291=CARTESIAN_POINT('Ctrl Pts',(16.7752912625975,20.0142117292613,-12.5386052246321));
#94292=CARTESIAN_POINT('Ctrl Pts',(16.7479923079759,19.9476406135874,-12.5342935179843));
#94293=CARTESIAN_POINT('Ctrl Pts',(16.7240840285397,19.8796585609645,-12.5299818113365));
#94294=CARTESIAN_POINT('Ctrl Pts',(16.7037024934053,19.8106507606227,-12.5256701046887));
#94295=CARTESIAN_POINT('Ctrl Pts',(16.6833204782337,19.7416413349709,-12.5213582964891));
#94296=CARTESIAN_POINT('Ctrl Pts',(16.6664655033664,19.6716065941827,-12.5170464882896));
#94297=CARTESIAN_POINT('Ctrl Pts',(16.6532233605847,19.6009456075705,-12.5127346800901));
#94298=CARTESIAN_POINT('Ctrl Pts',(16.6399664562209,19.5302058521387,-12.5084180653338));
#94299=CARTESIAN_POINT('Ctrl Pts',(16.630330506581,19.4588389489556,-12.5041014505775));
#94300=CARTESIAN_POINT('Ctrl Pts',(16.6243497245844,19.387251852299,-12.4997848358212));
#94301=CARTESIAN_POINT('Ctrl Pts',(16.6193948377084,19.3279442289965,-12.4962086583554));
#94302=CARTESIAN_POINT('Ctrl Pts',(16.6169477636251,19.2684857254403,-12.4926324808896));
#94303=CARTESIAN_POINT('Ctrl Pts',(16.6170008459317,19.2091074688849,-12.4890563034237));
#94304=CARTESIAN_POINT('Ctrl Pts',(16.6163526568764,19.2091064841458,-12.4890562790225));
#94305=CARTESIAN_POINT('Ctrl Pts',(16.6150299493055,19.0661177741218,-12.4804472042752));
#94306=CARTESIAN_POINT('Ctrl Pts',(16.637935879823,18.8192068412717,-12.4655558028099));
#94307=CARTESIAN_POINT('Ctrl Pts',(16.7071054573079,18.5818111963998,-12.4506644013445));
#94308=CARTESIAN_POINT('Ctrl Pts',(16.7437496504382,18.4842640742323,-12.4443820746265));
#94309=CARTESIAN_POINT('Origin',(18.734,19.211,0.));
#94310=CARTESIAN_POINT('',(16.7454194497538,18.4848895434008,-11.642549296791));
#94311=CARTESIAN_POINT('',(16.745419450367,18.4848895417216,-11.8674650022761));
#94312=CARTESIAN_POINT('',(16.7454194503191,18.4848895418526,0.));
#94313=CARTESIAN_POINT('',(16.6170009281725,19.212592427459,-11.9120627660338));
#94314=CARTESIAN_POINT('Ctrl Pts',(16.745419450367,18.4848895417216,-11.8674650022761));
#94315=CARTESIAN_POINT('Ctrl Pts',(16.7321284697392,18.5212892179149,-11.8699796928237));
#94316=CARTESIAN_POINT('Ctrl Pts',(16.7198387402319,18.5580487608643,-11.8724726230257));
#94317=CARTESIAN_POINT('Ctrl Pts',(16.7056938648529,18.6045673299265,-11.8755657071326));
#94318=CARTESIAN_POINT('Ctrl Pts',(16.7028893298231,18.6140277968553,-11.8761915999689));
#94319=CARTESIAN_POINT('Ctrl Pts',(16.6846213657658,18.6772699474235,-11.8803545196368));
#94320=CARTESIAN_POINT('Ctrl Pts',(16.6712285045199,18.7316303769976,-11.8838303722935));
#94321=CARTESIAN_POINT('Ctrl Pts',(16.6575927178034,18.7982452759099,-11.8879694743463));
#94322=CARTESIAN_POINT('Ctrl Pts',(16.6552811518111,18.810049101049,-11.8886984089892));
#94323=CARTESIAN_POINT('Ctrl Pts',(16.6516247957419,18.8296021107529,-11.8898986170216));
#94324=CARTESIAN_POINT('Ctrl Pts',(16.6502223883534,18.8373401158341,-11.8903717176368));
#94325=CARTESIAN_POINT('Ctrl Pts',(16.647762557358,18.851357294918,-11.891225390359));
#94326=CARTESIAN_POINT('Ctrl Pts',(16.6466902893433,18.857633737363,-11.8916064304635));
#94327=CARTESIAN_POINT('Ctrl Pts',(16.6446635453822,18.8698283232991,-11.892344452161));
#94328=CARTESIAN_POINT('Ctrl Pts',(16.6437058581411,18.875745864719,-11.8927015323105));
#94329=CARTESIAN_POINT('Ctrl Pts',(16.6416603294046,18.8887347544387,-11.8934830469093));
#94330=CARTESIAN_POINT('Ctrl Pts',(16.6405831710185,18.895807729015,-11.8939071403275));
#94331=CARTESIAN_POINT('Ctrl Pts',(16.6380228019412,18.9132122853069,-11.8949471700198));
#94332=CARTESIAN_POINT('Ctrl Pts',(16.636580092012,18.9235497030916,-11.8955618303798));
#94333=CARTESIAN_POINT('Ctrl Pts',(16.6230153970491,19.0262892828788,-11.9016413772041));
#94334=CARTESIAN_POINT('Ctrl Pts',(16.616930382029,19.1193894136381,-11.9069087404323));
#94335=CARTESIAN_POINT('Ctrl Pts',(16.6170006007779,19.2125948959813,-11.9120634735223));
#94336=CARTESIAN_POINT('Ctrl Pts',(16.6170005988961,19.2125923962176,-11.9120633352727));
#94337=CARTESIAN_POINT('Ctrl Pts',(16.6171096431973,19.3575605377985,-11.9200808075036));
#94338=CARTESIAN_POINT('Ctrl Pts',(16.6321085830719,19.5021326107325,-11.9277753928028));
#94339=CARTESIAN_POINT('Ctrl Pts',(16.6753598874925,19.7091047616055,-11.9395052990425));
#94340=CARTESIAN_POINT('Ctrl Pts',(16.6920125343409,19.7734881594003,-11.9432642931686));
#94341=CARTESIAN_POINT('Ctrl Pts',(16.7155919333298,19.8496660885941,-11.9479594196532));
#94342=CARTESIAN_POINT('Ctrl Pts',(16.719639492168,19.862319599458,-11.9487476794528));
#94343=CARTESIAN_POINT('Ctrl Pts',(16.72545184711,19.8799176825956,-11.9498567722796));
#94344=CARTESIAN_POINT('Ctrl Pts',(16.7271164455099,19.8848953523641,-11.9501719199984));
#94345=CARTESIAN_POINT('Ctrl Pts',(16.7299780585381,19.8933478330375,-11.9507095947849));
#94346=CARTESIAN_POINT('Ctrl Pts',(16.731165656707,19.8968258526719,-11.9509315671638));
#94347=CARTESIAN_POINT('Ctrl Pts',(16.7334554379233,19.9034750727794,-11.9513573594417));
#94348=CARTESIAN_POINT('Ctrl Pts',(16.7345561151745,19.9066467654954,-11.9515610853202));
#94349=CARTESIAN_POINT('Ctrl Pts',(16.7374837715901,19.9150187002132,-11.9521004549986));
#94350=CARTESIAN_POINT('Ctrl Pts',(16.7393235090342,19.9202144071966,-11.9524368465735));
#94351=CARTESIAN_POINT('Ctrl Pts',(16.7458814187719,19.9385076035979,-11.9536269110739));
#94352=CARTESIAN_POINT('Ctrl Pts',(16.7507083566868,19.9515653518591,-11.9544866873335));
#94353=CARTESIAN_POINT('Ctrl Pts',(16.8148892225599,20.1200575249106,-11.9657060977763));
#94354=CARTESIAN_POINT('Ctrl Pts',(16.8922334230719,20.2680061410319,-11.9768935262057));
#94355=CARTESIAN_POINT('Ctrl Pts',(17.0313948872008,20.4716635449461,-11.9930979087352));
#94356=CARTESIAN_POINT('Ctrl Pts',(17.080435770946,20.5353353551139,-11.9983095844323));
#94357=CARTESIAN_POINT('Ctrl Pts',(17.1587118285267,20.6258155367969,-12.0058900509515));
#94358=CARTESIAN_POINT('Ctrl Pts',(17.1852688175454,20.6548378940967,-12.0083516948774));
#94359=CARTESIAN_POINT('Ctrl Pts',(17.2310760798334,20.7021784255388,-12.0124188401085));
#94360=CARTESIAN_POINT('Ctrl Pts',(17.2498894116488,20.7209037282837,-12.0140420857559));
#94361=CARTESIAN_POINT('Ctrl Pts',(17.2761175036621,20.7460450992286,-12.0162427142381));
#94362=CARTESIAN_POINT('Ctrl Pts',(17.2832314096017,20.7527701942719,-12.0168335153521));
#94363=CARTESIAN_POINT('Ctrl Pts',(17.2947498907459,20.7635088161135,-12.0177804811171));
#94364=CARTESIAN_POINT('Ctrl Pts',(17.2991251469649,20.7675534550262,-12.018137979877));
#94365=CARTESIAN_POINT('Ctrl Pts',(17.3082764796628,20.7759418907548,-12.0188811854216));
#94366=CARTESIAN_POINT('Ctrl Pts',(17.3130554731019,20.7802824254369,-12.0192667512797));
#94367=CARTESIAN_POINT('Ctrl Pts',(17.3241346827433,20.7902530434893,-12.0201547977397));
#94368=CARTESIAN_POINT('Ctrl Pts',(17.3304489253187,20.795867430447,-12.0206566140765));
#94369=CARTESIAN_POINT('Ctrl Pts',(17.3475179863695,20.8108625826355,-12.0220017942487));
#94370=CARTESIAN_POINT('Ctrl Pts',(17.3583344437239,20.8201727531766,-12.0228422265579));
#94371=CARTESIAN_POINT('Ctrl Pts',(17.458578271993,20.9047072351699,-12.030524409898));
#94372=CARTESIAN_POINT('Ctrl Pts',(17.5540015251732,20.9725202664418,-12.0370493181345));
#94373=CARTESIAN_POINT('Ctrl Pts',(17.7945472526606,21.1151019582931,-12.0523574721807));
#94374=CARTESIAN_POINT('Ctrl Pts',(17.9436329802301,21.1816556906102,-12.0609576997701));
#94375=CARTESIAN_POINT('Ctrl Pts',(18.1298554940101,21.24022521602,-12.0721667263814));
#94376=CARTESIAN_POINT('Ctrl Pts',(18.1610814346634,21.2492614203661,-12.0740625626132));
#94377=CARTESIAN_POINT('Ctrl Pts',(18.1994995612107,21.2594263934635,-12.0764287290479));
#94378=CARTESIAN_POINT('Ctrl Pts',(18.2065074413095,21.2612421821793,-12.0768617015604));
#94379=CARTESIAN_POINT('Ctrl Pts',(18.2175078875264,21.2640323394769,-12.0775436736093));
#94380=CARTESIAN_POINT('Ctrl Pts',(18.2214942884731,21.2650311059421,-12.0777912874916));
#94381=CARTESIAN_POINT('Ctrl Pts',(18.2289509060658,21.2668762539518,-12.0782553870358));
#94382=CARTESIAN_POINT('Ctrl Pts',(18.232420365192,21.2677254625099,-12.0784717073496));
#94383=CARTESIAN_POINT('Ctrl Pts',(18.2403449178979,21.2696438863852,-12.0789666632021));
#94384=CARTESIAN_POINT('Ctrl Pts',(18.2448013281175,21.2707074184343,-12.0792456206439));
#94385=CARTESIAN_POINT('Ctrl Pts',(18.2585093924889,21.2739318809382,-12.0801055216055));
#94386=CARTESIAN_POINT('Ctrl Pts',(18.2677720208626,21.2760449697184,-12.0806891046106));
#94387=CARTESIAN_POINT('Ctrl Pts',(18.3518861181507,21.2946392113131,-12.0860096904517));
#94388=CARTESIAN_POINT('Ctrl Pts',(18.4275592304074,21.3071046800085,-12.0909455788181));
#94389=CARTESIAN_POINT('Ctrl Pts',(18.654447904586,21.3319308530719,-12.1058777259792));
#94390=CARTESIAN_POINT('Ctrl Pts',(18.8065177145713,21.3321847429283,-12.1160236107794));
#94391=CARTESIAN_POINT('Ctrl Pts',(19.0322519158724,21.3082396384638,-12.130611715981));
#94392=CARTESIAN_POINT('Ctrl Pts',(19.1067209252473,21.2962936463815,-12.135353870288));
#94393=CARTESIAN_POINT('Ctrl Pts',(19.198829694997,21.2764243504998,-12.1411265578811));
#94394=CARTESIAN_POINT('Ctrl Pts',(19.2172042100089,21.2722030759988,-12.1422736217243));
#94395=CARTESIAN_POINT('Ctrl Pts',(19.2438390872505,21.2657083542146,-12.1439302146524));
#94396=CARTESIAN_POINT('Ctrl Pts',(19.252145518692,21.2636294211552,-12.1444459728751));
#94397=CARTESIAN_POINT('Ctrl Pts',(19.2666870459439,21.2598960733974,-12.1453474133604));
#94398=CARTESIAN_POINT('Ctrl Pts',(19.2729275758728,21.2582634607915,-12.1457337942411));
#94399=CARTESIAN_POINT('Ctrl Pts',(19.2850308851751,21.2550378840272,-12.1464822815137));
#94400=CARTESIAN_POINT('Ctrl Pts',(19.2908944548695,21.2534481572551,-12.1468444884299));
#94401=CARTESIAN_POINT('Ctrl Pts',(19.3048955079425,21.2495874259188,-12.1477084383598));
#94402=CARTESIAN_POINT('Ctrl Pts',(19.3130264400135,21.247292896175,-12.1482094135657));
#94403=CARTESIAN_POINT('Ctrl Pts',(19.3423181631736,21.2388372077739,-12.1500116421698));
#94404=CARTESIAN_POINT('Ctrl Pts',(19.3633966292388,21.2323942380903,-12.1513037236844));
#94405=CARTESIAN_POINT('Ctrl Pts',(19.5615602018388,21.1684220296981,-12.1634154528012));
#94406=CARTESIAN_POINT('Ctrl Pts',(19.7304240961551,21.0880993238893,-12.1733718258654));
#94407=CARTESIAN_POINT('Ctrl Pts',(19.9535081067484,20.9432959069571,-12.1878722757483));
#94408=CARTESIAN_POINT('Ctrl Pts',(20.0178898790075,20.8961332069108,-12.1922591821868));
#94409=CARTESIAN_POINT('Ctrl Pts',(20.1071884375814,20.8226243594735,-12.1988759154432));
#94410=CARTESIAN_POINT('Ctrl Pts',(20.1343368086098,20.799091948806,-12.2009656715114));
#94411=CARTESIAN_POINT('Ctrl Pts',(20.1663822772901,20.7698539574843,-12.2035472600936));
#94412=CARTESIAN_POINT('Ctrl Pts',(20.171866336212,20.7647969765995,-12.2039932552835));
#94413=CARTESIAN_POINT('Ctrl Pts',(20.180365229202,20.7568764219995,-12.2046912189808));
#94414=CARTESIAN_POINT('Ctrl Pts',(20.1833986098913,20.7540327142679,-12.2049416927658));
#94415=CARTESIAN_POINT('Ctrl Pts',(20.1890179701563,20.748733534535,-12.2054082753903));
#94416=CARTESIAN_POINT('Ctrl Pts',(20.1916061301188,20.7462804582696,-12.2056242011531));
#94417=CARTESIAN_POINT('Ctrl Pts',(20.1974553340714,20.7407084190773,-12.2061145178176));
#94418=CARTESIAN_POINT('Ctrl Pts',(20.2007125948627,20.7375855774955,-12.2063892069038));
#94419=CARTESIAN_POINT('Ctrl Pts',(20.209099549725,20.7294931114919,-12.2071006915996));
#94420=CARTESIAN_POINT('Ctrl Pts',(20.2142140748927,20.7245079452776,-12.2075386567639));
#94421=CARTESIAN_POINT('Ctrl Pts',(20.2455220078266,20.693681387191,-12.210244313257));
#94422=CARTESIAN_POINT('Ctrl Pts',(20.2710615509035,20.6671882734104,-12.2125585183994));
#94423=CARTESIAN_POINT('Ctrl Pts',(20.4110382717863,20.5141986494772,-12.2257933979694));
#94424=CARTESIAN_POINT('Ctrl Pts',(20.5105487228058,20.3748994255009,-12.2373030417796));
#94425=CARTESIAN_POINT('Ctrl Pts',(20.6378804230543,20.1415880144799,-12.2545747517269));
#94426=CARTESIAN_POINT('Ctrl Pts',(20.6778077626523,20.0550203373955,-12.2606236815293));
#94427=CARTESIAN_POINT('Ctrl Pts',(20.7193968869128,19.9460815808388,-12.2677862145821));
#94428=CARTESIAN_POINT('Ctrl Pts',(20.7267165667087,19.9260010254396,-12.2690888545118));
#94429=CARTESIAN_POINT('Ctrl Pts',(20.7366870790697,19.8973050180554,-12.2709260702917));
#94430=CARTESIAN_POINT('Ctrl Pts',(20.7395887362517,19.8887786802632,-12.2714689368068));
#94431=CARTESIAN_POINT('Ctrl Pts',(20.7444988638096,19.8740429123714,-12.2724020347105));
#94432=CARTESIAN_POINT('Ctrl Pts',(20.746533179379,19.867842285792,-12.2727931158146));
#94433=CARTESIAN_POINT('Ctrl Pts',(20.750372201096,19.8559556052995,-12.2735398881133));
#94434=CARTESIAN_POINT('Ctrl Pts',(20.7521816049166,19.8502711450222,-12.2738957308973));
#94435=CARTESIAN_POINT('Ctrl Pts',(20.756821661761,19.8354777876433,-12.2748185044937));
#94436=CARTESIAN_POINT('Ctrl Pts',(20.7596148434133,19.8263572078229,-12.2753842022615));
#94437=CARTESIAN_POINT('Ctrl Pts',(20.7689166512403,19.7952342630008,-12.277303881443));
#94438=CARTESIAN_POINT('Ctrl Pts',(20.7751293294765,19.7731446188228,-12.2786482176882));
#94439=CARTESIAN_POINT('Ctrl Pts',(20.825898967173,19.5806767085031,-12.2902153262119));
#94440=CARTESIAN_POINT('Ctrl Pts',(20.8493946346846,19.4054591659866,-12.2996809660499));
#94441=CARTESIAN_POINT('Ctrl Pts',(20.8516705394732,19.1427783830044,-12.3139756449634));
#94442=CARTESIAN_POINT('Ctrl Pts',(20.8471102895636,19.0562575131338,-12.3187160867395));
#94443=CARTESIAN_POINT('Ctrl Pts',(20.8329796080339,18.9327989813262,-12.3258117197912));
#94444=CARTESIAN_POINT('Ctrl Pts',(20.8276910922077,18.8954553657526,-12.3280024935771));
#94445=CARTESIAN_POINT('Ctrl Pts',(20.8201480559763,18.8508159871393,-12.3306961049287));
#94446=CARTESIAN_POINT('Ctrl Pts',(20.8188475968985,18.8433633201579,-12.3311483316482));
#94447=CARTESIAN_POINT('Ctrl Pts',(20.816766487635,18.8318031674425,-12.3318539409595));
#94448=CARTESIAN_POINT('Ctrl Pts',(20.8160135529639,18.8276906674528,-12.3321057753653));
#94449=CARTESIAN_POINT('Ctrl Pts',(20.814596239774,18.8200767486476,-12.3325735800166));
#94450=CARTESIAN_POINT('Ctrl Pts',(20.8139352000489,18.8165747670038,-12.3327893588814));
#94451=CARTESIAN_POINT('Ctrl Pts',(20.8124228702988,18.8086724472087,-12.3332776537651));
#94452=CARTESIAN_POINT('Ctrl Pts',(20.81156645218,18.8042731586955,-12.333550457455));
#94453=CARTESIAN_POINT('Ctrl Pts',(20.8090037942633,18.791328474557,-12.3343559463221));
#94454=CARTESIAN_POINT('Ctrl Pts',(20.8072587783973,18.7827909771194,-12.3348907647034));
#94455=CARTESIAN_POINT('Ctrl Pts',(20.7944756120108,18.722159673948,-12.3387131405802));
#94456=CARTESIAN_POINT('Ctrl Pts',(20.7815289897598,18.670492260103,-12.3420974229617));
#94457=CARTESIAN_POINT('Ctrl Pts',(20.7620074593084,18.6034222527144,-12.3466116864115));
#94458=CARTESIAN_POINT('Ctrl Pts',(20.7571773535687,18.5875271862588,-12.3476906473172));
#94459=CARTESIAN_POINT('Ctrl Pts',(20.7477278573139,18.5576971662977,-12.3497308935988));
#94460=CARTESIAN_POINT('Ctrl Pts',(20.7431495701874,18.5437500695347,-12.3506912143554));
#94461=CARTESIAN_POINT('Ctrl Pts',(20.6967208145958,18.4071233431848,-12.3601554002246));
#94462=CARTESIAN_POINT('Ctrl Pts',(20.643827624164,18.2884747834949,-12.3688036312122));
#94463=CARTESIAN_POINT('Ctrl Pts',(20.5373339064651,18.098601224779,-12.3828978167145));
#94464=CARTESIAN_POINT('Ctrl Pts',(20.4895004456536,18.0245490779237,-12.3884735194934));
#94465=CARTESIAN_POINT('Ctrl Pts',(20.4250118794719,17.9371915185115,-12.3951371656135));
#94466=CARTESIAN_POINT('Ctrl Pts',(20.4125977907129,17.9208764681488,-12.3963859236246));
#94467=CARTESIAN_POINT('Ctrl Pts',(20.3944833488965,17.8977740131278,-12.3981608747712));
#94468=CARTESIAN_POINT('Ctrl Pts',(20.3889746155053,17.8908384680965,-12.3986946130581));
#94469=CARTESIAN_POINT('Ctrl Pts',(20.3793484338425,17.8788739663909,-12.3996169764498));
#94470=CARTESIAN_POINT('Ctrl Pts',(20.3752510843287,17.8738290618553,-12.4000063998237));
#94471=CARTESIAN_POINT('Ctrl Pts',(20.3673276039515,17.8641644803954,-12.4007534303614));
#94472=CARTESIAN_POINT('Ctrl Pts',(20.3635049492072,17.8595420464004,-12.4011111726863));
#94473=CARTESIAN_POINT('Ctrl Pts',(20.3534379427263,17.8474736224625,-12.4020464007615));
#94474=CARTESIAN_POINT('Ctrl Pts',(20.3471618317371,17.8400542162463,-12.4026225856986));
#94475=CARTESIAN_POINT('Ctrl Pts',(20.325195478112,17.8144460449859,-12.4046158489699));
#94476=CARTESIAN_POINT('Ctrl Pts',(20.3092465616662,17.7964808809792,-12.4060222392967));
#94477=CARTESIAN_POINT('Ctrl Pts',(20.1927354910093,17.6696557498313,-12.4160193822394));
#94478=CARTESIAN_POINT('Ctrl Pts',(20.0812918925884,17.5713468127318,-12.4241001588517));
#94479=CARTESIAN_POINT('Ctrl Pts',(19.9229286085026,17.4587841409114,-12.4346515884927));
#94480=CARTESIAN_POINT('Ctrl Pts',(19.8845151478869,17.4333255505874,-12.4371511184435));
#94481=CARTESIAN_POINT('Ctrl Pts',(19.7845337156379,17.3716616922227,-12.4435769042513));
#94482=CARTESIAN_POINT('Ctrl Pts',(19.721912533718,17.3372834331545,-12.4475273896887));
#94483=CARTESIAN_POINT('Ctrl Pts',(19.6274697117914,17.291487528235,-12.4535470183183));
#94484=CARTESIAN_POINT('Ctrl Pts',(19.596917157227,17.2775600736383,-12.4555036208632));
#94485=CARTESIAN_POINT('Ctrl Pts',(19.5593255912544,17.2614923387313,-12.4579373551384));
#94486=CARTESIAN_POINT('Ctrl Pts',(19.5525880771511,17.2586537168506,-12.4583745682869));
#94487=CARTESIAN_POINT('Ctrl Pts',(19.5420260971823,17.2542680701593,-12.4590617496848));
#94488=CARTESIAN_POINT('Ctrl Pts',(19.5382115089865,17.2526971972823,-12.4593102971578));
#94489=CARTESIAN_POINT('Ctrl Pts',(19.5310875593136,17.2497878324102,-12.4597751937771));
#94490=CARTESIAN_POINT('Ctrl Pts',(19.5277793955357,17.2484465576455,-12.4599913717436));
#94491=CARTESIAN_POINT('Ctrl Pts',(19.5202392979072,17.2454116544916,-12.4604847515597));
#94492=CARTESIAN_POINT('Ctrl Pts',(19.5160052936139,17.2437233297185,-12.460762267312));
#94493=CARTESIAN_POINT('Ctrl Pts',(19.5049830520162,17.239369375471,-12.4614858655785));
#94494=CARTESIAN_POINT('Ctrl Pts',(19.4981865003339,17.2367251520474,-12.4619331834344));
#94495=CARTESIAN_POINT('Ctrl Pts',(19.4548264452209,17.2201132058259,-12.4647935106258));
#94496=CARTESIAN_POINT('Ctrl Pts',(19.4178976208762,17.2071276018675,-12.4672591479848));
#94497=CARTESIAN_POINT('Ctrl Pts',(19.368876677719,17.1914027538968,-12.4705515730435));
#94498=CARTESIAN_POINT('Ctrl Pts',(19.3570878125481,17.1877345701858,-12.4713448221732));
#94499=CARTESIAN_POINT('Ctrl Pts',(19.3221513500614,17.1771981510138,-12.4736986868448));
#94500=CARTESIAN_POINT('Ctrl Pts',(19.2989179713522,17.1706226831521,-12.4752679828094));
#94501=CARTESIAN_POINT('Ctrl Pts',(19.136219586817,17.1275679421086,-12.4862637304607));
#94502=CARTESIAN_POINT('Ctrl Pts',(18.9934447957794,17.1050172893108,-12.4959108505562));
#94503=CARTESIAN_POINT('Ctrl Pts',(18.7877688675211,17.0937805088541,-12.5092191007373));
#94504=CARTESIAN_POINT('Ctrl Pts',(18.725928863084,17.0931129746347,-12.5131506922479));
#94505=CARTESIAN_POINT('Ctrl Pts',(18.6269048287152,17.0963823389101,-12.5193243150439));
#94506=CARTESIAN_POINT('Ctrl Pts',(18.589703425803,17.0985947349766,-12.5216162621416));
#94507=CARTESIAN_POINT('Ctrl Pts',(18.5414838681116,17.1027423008144,-12.5245533575229));
#94508=CARTESIAN_POINT('Ctrl Pts',(18.5303974165945,17.1037840683346,-12.5252263380837));
#94509=CARTESIAN_POINT('Ctrl Pts',(18.5123855124175,17.1056200820047,-12.526316088961));
#94510=CARTESIAN_POINT('Ctrl Pts',(18.5054549622964,17.1063611360252,-12.5267345251576));
#94511=CARTESIAN_POINT('Ctrl Pts',(18.4921372978715,17.1078516962115,-12.5275369491177));
#94512=CARTESIAN_POINT('Ctrl Pts',(18.4857497012345,17.108596103271,-12.5279210927996));
#94513=CARTESIAN_POINT('Ctrl Pts',(18.4711367115343,17.1103666195087,-12.528798286207));
#94514=CARTESIAN_POINT('Ctrl Pts',(18.4629137212387,17.1114119594293,-12.5292907239928));
#94515=CARTESIAN_POINT('Ctrl Pts',(18.4410945113366,17.1143160276475,-12.5305943799195));
#94516=CARTESIAN_POINT('Ctrl Pts',(18.4275097236942,17.116258720279,-12.5314029463139));
#94517=CARTESIAN_POINT('Ctrl Pts',(18.3247120659353,17.1319807427865,-12.5374997844465));
#94518=CARTESIAN_POINT('Ctrl Pts',(18.2364379517191,17.1513222199464,-12.5426055671439));
#94519=CARTESIAN_POINT('Ctrl Pts',(18.0155892138936,17.2147454531445,-12.5553255416308));
#94520=CARTESIAN_POINT('Ctrl Pts',(17.8856584964277,17.2664020691091,-12.5627450038856));
#94521=CARTESIAN_POINT('Ctrl Pts',(17.7126395441167,17.3558533749178,-12.5735037395324));
#94522=CARTESIAN_POINT('Ctrl Pts',(17.6645406028387,17.3831592167064,-12.5766018451786));
#94523=CARTESIAN_POINT('Ctrl Pts',(17.5933680159443,17.4273355104765,-12.5814337294784));
#94524=CARTESIAN_POINT('Ctrl Pts',(17.5694739196579,17.4428430040043,-12.5831003750124));
#94525=CARTESIAN_POINT('Ctrl Pts',(17.5401543114251,17.4627237960453,-12.5852109951811));
#94526=CARTESIAN_POINT('Ctrl Pts',(17.5344266221051,17.466648853745,-12.58562648726));
#94527=CARTESIAN_POINT('Ctrl Pts',(17.5253935807098,17.4729045251356,-12.586286969709));
#94528=CARTESIAN_POINT('Ctrl Pts',(17.5220753618901,17.4752165954805,-12.5865307152054));
#94529=CARTESIAN_POINT('Ctrl Pts',(17.5158296036695,17.4795951581254,-12.5869916705161));
#94530=CARTESIAN_POINT('Ctrl Pts',(17.512900678641,17.48165958018,-12.587208739687));
#94531=CARTESIAN_POINT('Ctrl Pts',(17.5062161283549,17.4863965638748,-12.587706208314));
#94532=CARTESIAN_POINT('Ctrl Pts',(17.5024639856418,17.4890739586793,-12.5879869371815));
#94533=CARTESIAN_POINT('Ctrl Pts',(17.4925254489283,17.4962148433087,-12.5887344254519));
#94534=CARTESIAN_POINT('Ctrl Pts',(17.4863544516233,17.500699507057,-12.5892025899524));
#94535=CARTESIAN_POINT('Ctrl Pts',(17.4432974580955,17.5323474527857,-12.5924967257349));
#94536=CARTESIAN_POINT('Ctrl Pts',(17.407280202645,17.5606663014199,-12.5953947608523));
#94537=CARTESIAN_POINT('Ctrl Pts',(17.3434298709737,17.6143106269932,-12.6007561933977));
#94538=CARTESIAN_POINT('Ctrl Pts',(17.315297263426,17.6392542963525,-12.6032035501016));
#94539=CARTESIAN_POINT('Ctrl Pts',(17.1921807784063,17.7544145681658,-12.6142536644186));
#94540=CARTESIAN_POINT('Ctrl Pts',(17.1050207995226,17.8525898696697,-12.6229968670819));
#94541=CARTESIAN_POINT('Ctrl Pts',(16.9752027213444,18.0294209688657,-12.6372013371042));
#94542=CARTESIAN_POINT('Ctrl Pts',(16.9274171728916,18.1038600867,-12.6427967365363));
#94543=CARTESIAN_POINT('Ctrl Pts',(16.8744284151348,18.1990196298712,-12.6494812445963));
#94544=CARTESIAN_POINT('Ctrl Pts',(16.8646987222113,18.2171068828746,-12.6507322979998));
#94545=CARTESIAN_POINT('Ctrl Pts',(16.8511486118679,18.2431992926252,-12.6525099078202));
#94546=CARTESIAN_POINT('Ctrl Pts',(16.8471131308596,18.2510908867055,-12.653044040467));
#94547=CARTESIAN_POINT('Ctrl Pts',(16.8402042040713,18.26481358278,-12.6539668662221));
#94548=CARTESIAN_POINT('Ctrl Pts',(16.8373078572203,18.2706329600688,-12.6543563598096));
#94549=CARTESIAN_POINT('Ctrl Pts',(16.8317911219144,18.281846436332,-12.6551033731214));
#94550=CARTESIAN_POINT('Ctrl Pts',(16.8291667639027,18.2872385023488,-12.6554610287311));
#94551=CARTESIAN_POINT('Ctrl Pts',(16.8223533113959,18.3013900762796,-12.6563956933988));
#94552=CARTESIAN_POINT('Ctrl Pts',(16.8182014751491,18.3101674448976,-12.65697140473));
#94553=CARTESIAN_POINT('Ctrl Pts',(16.8040088660262,18.340713888129,-12.6589613795846));
#94554=CARTESIAN_POINT('Ctrl Pts',(16.7942773401895,18.3626252210065,-12.6603650026611));
#94555=CARTESIAN_POINT('Ctrl Pts',(16.770898167933,18.417771972556,-12.6638421750932));
#94556=CARTESIAN_POINT('Ctrl Pts',(16.7577281090364,18.4511801383449,-12.6658990859603));
#94557=CARTESIAN_POINT('Ctrl Pts',(16.7454195353148,18.4848893090773,-12.6679318638109));
#94558=CARTESIAN_POINT('',(16.6141771432254,19.2120774369074,-11.6890562790225));
#94559=CARTESIAN_POINT('Ctrl Pts',(16.7437496504382,18.4842640742323,-12.4443820746265));
#94560=CARTESIAN_POINT('Ctrl Pts',(16.9543734431303,17.9235819283861,-12.4082724657841));
#94561=CARTESIAN_POINT('Ctrl Pts',(17.94829019586,16.8917270960979,-12.329770921381));
#94562=CARTESIAN_POINT('Ctrl Pts',(20.2082246499765,17.1878857088602,-12.2088774414178));
#94563=CARTESIAN_POINT('Ctrl Pts',(21.2330887962208,19.3555162351247,-12.0817016347362));
#94564=CARTESIAN_POINT('Ctrl Pts',(19.9651940828767,21.3905620853514,-11.9545258280549));
#94565=CARTESIAN_POINT('Ctrl Pts',(17.567755215016,21.4259950011477,-11.8273500213734));
#94566=CARTESIAN_POINT('Ctrl Pts',(16.6440838354548,20.0366853275688,-11.7388601716959));
#94567=CARTESIAN_POINT('Ctrl Pts',(16.613796038846,19.2734660709366,-11.692762257579));
#94568=CARTESIAN_POINT('Ctrl Pts',(16.6141771432254,19.2120774369074,-11.6890562790225));
#94569=CARTESIAN_POINT('Ctrl Pts',(16.6170002227512,19.2119711480246,-11.6906772989821));
#94570=CARTESIAN_POINT('Ctrl Pts',(16.6169205026538,19.0381897839503,-11.6794990057181));
#94571=CARTESIAN_POINT('Ctrl Pts',(16.6382377399725,18.865048996398,-11.6677742008829));
#94572=CARTESIAN_POINT('Ctrl Pts',(16.6953336165312,18.6371881017047,-11.6526052839768));
#94573=CARTESIAN_POINT('Ctrl Pts',(16.7127403586391,18.5785988026368,-11.6487214519702));
#94574=CARTESIAN_POINT('Ctrl Pts',(16.7368041306635,18.5088181354777,-11.6441232612583));
#94575=CARTESIAN_POINT('Ctrl Pts',(16.7410579839532,18.4968341807256,-11.6433345260294));
#94576=CARTESIAN_POINT('Ctrl Pts',(16.7454194497538,18.4848895434008,-11.642549296791));
#94577=CARTESIAN_POINT('Origin',(18.734,19.211,0.));
#94578=CARTESIAN_POINT('',(16.7454194500511,18.4848895425866,-10.8441190257052));
#94579=CARTESIAN_POINT('',(16.7454194505824,18.4848895411316,-11.0644158872188));
#94580=CARTESIAN_POINT('',(16.7454194503191,18.4848895418526,0.));
#94581=CARTESIAN_POINT('Ctrl Pts',(16.7454194505824,18.4848895411316,-11.0644158872188));
#94582=CARTESIAN_POINT('Ctrl Pts',(16.7100155209546,18.5818493975431,-11.0708123982825));
#94583=CARTESIAN_POINT('Ctrl Pts',(16.6817531128539,18.681261479843,-11.0775606724488));
#94584=CARTESIAN_POINT('Ctrl Pts',(16.6317924842058,18.922881279888,-11.0938351315304));
#94585=CARTESIAN_POINT('Ctrl Pts',(16.6170952308513,19.0660441061833,-11.103353731068));
#94586=CARTESIAN_POINT('Ctrl Pts',(16.6169595358832,19.2715966104105,-11.1164063514006));
#94587=CARTESIAN_POINT('Ctrl Pts',(16.6196417425651,19.3335670533862,-11.1202673935233));
#94588=CARTESIAN_POINT('Ctrl Pts',(16.6261219959195,19.4077067085304,-11.1248001812546));
#94589=CARTESIAN_POINT('Ctrl Pts',(16.6273121369466,19.4200680923591,-11.1255530928494));
#94590=CARTESIAN_POINT('Ctrl Pts',(16.6294460864631,19.4403590520909,-11.1267844640882));
#94591=CARTESIAN_POINT('Ctrl Pts',(16.630326098816,19.448294900835,-11.1272649195133));
#94592=CARTESIAN_POINT('Ctrl Pts',(16.6319896971689,19.4625598422829,-11.1281265638762));
#94593=CARTESIAN_POINT('Ctrl Pts',(16.6327570213205,19.4688907004645,-11.1285082603374));
#94594=CARTESIAN_POINT('Ctrl Pts',(16.6344530088735,19.4823732466887,-11.1293196760289));
#94595=CARTESIAN_POINT('Ctrl Pts',(16.635389634705,19.489523865437,-11.1297491389087));
#94596=CARTESIAN_POINT('Ctrl Pts',(16.6380125560209,19.5087836565671,-11.1309035772139));
#94597=CARTESIAN_POINT('Ctrl Pts',(16.6397672554953,19.5208833534279,-11.131626385958));
#94598=CARTESIAN_POINT('Ctrl Pts',(16.6490971429036,19.5815156080685,-11.1352369209254));
#94599=CARTESIAN_POINT('Ctrl Pts',(16.6582553385621,19.6297915850873,-11.1380741281951));
#94600=CARTESIAN_POINT('Ctrl Pts',(16.6895710865478,19.768345710885,-11.1461497711089));
#94601=CARTESIAN_POINT('Ctrl Pts',(16.7160033333925,19.8575410347184,-11.1512603757036));
#94602=CARTESIAN_POINT('Ctrl Pts',(16.8056500760732,20.1001682217777,-11.1653488990541));
#94603=CARTESIAN_POINT('Ctrl Pts',(16.8811330610567,20.2483141341045,-11.1741493464689));
#94604=CARTESIAN_POINT('Ctrl Pts',(16.9808577988162,20.3977505844248,-11.1847107227762));
#94605=CARTESIAN_POINT('Ctrl Pts',(16.98873445628,20.4093040873631,-11.1855393832611));
#94606=CARTESIAN_POINT('Ctrl Pts',(16.9998805489716,20.4253101852528,-11.1867056854588));
#94607=CARTESIAN_POINT('Ctrl Pts',(17.0030540294999,20.429829578773,-11.1870370549439));
#94608=CARTESIAN_POINT('Ctrl Pts',(17.0081863109764,20.4370780543811,-11.1875719354958));
#94609=CARTESIAN_POINT('Ctrl Pts',(17.0101340133915,20.4398150163902,-11.1877746886095));
#94610=CARTESIAN_POINT('Ctrl Pts',(17.0142251821318,20.4455351634391,-11.1882001112914));
#94611=CARTESIAN_POINT('Ctrl Pts',(17.0163699007564,20.4485174081177,-11.1884228701987));
#94612=CARTESIAN_POINT('Ctrl Pts',(17.0215923833213,20.4557395728477,-11.1889646379422));
#94613=CARTESIAN_POINT('Ctrl Pts',(17.0246781354243,20.4599736633754,-11.1892841947015));
#94614=CARTESIAN_POINT('Ctrl Pts',(17.0356087267315,20.4748556096623,-11.1904140905413));
#94615=CARTESIAN_POINT('Ctrl Pts',(17.0435374119241,20.4854411077792,-11.1912299669469));
#94616=CARTESIAN_POINT('Ctrl Pts',(17.0915650921809,20.5483255707599,-11.1961467131398));
#94617=CARTESIAN_POINT('Ctrl Pts',(17.1339858129166,20.5987986288466,-11.2003844459875));
#94618=CARTESIAN_POINT('Ctrl Pts',(17.2439182046635,20.7178479316795,-11.2109620835965));
#94619=CARTESIAN_POINT('Ctrl Pts',(17.3138862261073,20.7839625368012,-11.2173577552389));
#94620=CARTESIAN_POINT('Ctrl Pts',(17.4967378702986,20.9345654833649,-11.2329412957291));
#94621=CARTESIAN_POINT('Ctrl Pts',(17.6140380995269,21.0129972723151,-11.2419898342652));
#94622=CARTESIAN_POINT('Ctrl Pts',(17.7508858945676,21.0859346175174,-11.2514584834878));
#94623=CARTESIAN_POINT('Ctrl Pts',(17.7635632818766,21.09252750607,-11.2523264140155));
#94624=CARTESIAN_POINT('Ctrl Pts',(17.7838464437517,21.1028162423241,-11.2537006644079));
#94625=CARTESIAN_POINT('Ctrl Pts',(17.7914091180115,21.1065956603674,-11.2542099119544));
#94626=CARTESIAN_POINT('Ctrl Pts',(17.8047871230571,21.1131814104047,-11.2551052749282));
#94627=CARTESIAN_POINT('Ctrl Pts',(17.8105929944578,21.1160066121445,-11.2554920464123));
#94628=CARTESIAN_POINT('Ctrl Pts',(17.8226282448171,21.1217951507859,-11.2562901181425));
#94629=CARTESIAN_POINT('Ctrl Pts',(17.8288593712895,21.124754693894,-11.2567012829711));
#94630=CARTESIAN_POINT('Ctrl Pts',(17.8448911769946,21.1322733632655,-11.2577540212421));
#94631=CARTESIAN_POINT('Ctrl Pts',(17.8547125856237,21.1367880166358,-11.2583940532195));
#94632=CARTESIAN_POINT('Ctrl Pts',(17.8958499820366,21.1553175219463,-11.2610549434631));
#94633=CARTESIAN_POINT('Ctrl Pts',(17.9274707809677,21.1686457530066,-11.2630522679164));
#94634=CARTESIAN_POINT('Ctrl Pts',(18.0106938833782,21.2013654595668,-11.2681969654979));
#94635=CARTESIAN_POINT('Ctrl Pts',(18.0627550250274,21.2195211550232,-11.2713049371841));
#94636=CARTESIAN_POINT('Ctrl Pts',(18.2200495712485,21.267575302397,-11.2804500677529));
#94637=CARTESIAN_POINT('Ctrl Pts',(18.326951961139,21.2913749168322,-11.2863384996509));
#94638=CARTESIAN_POINT('Ctrl Pts',(18.4810914173601,21.3133495800491,-11.2948153811085));
#94639=CARTESIAN_POINT('Ctrl Pts',(18.5271698631718,21.3183816819776,-11.2973493723591));
#94640=CARTESIAN_POINT('Ctrl Pts',(18.5947048982484,21.3235206463984,-11.3011064844839));
#94641=CARTESIAN_POINT('Ctrl Pts',(18.6160578680894,21.3248202897957,-11.302300710048));
#94642=CARTESIAN_POINT('Ctrl Pts',(18.6892274552065,21.328161630565,-11.3064251205685));
#94643=CARTESIAN_POINT('Ctrl Pts',(18.7410935464018,21.3286228862856,-11.3094038028982));
#94644=CARTESIAN_POINT('Ctrl Pts',(18.8015714079021,21.326939039566,-11.3129945970821));
#94645=CARTESIAN_POINT('Ctrl Pts',(18.8102216347434,21.3266450956905,-11.3135110055463));
#94646=CARTESIAN_POINT('Ctrl Pts',(18.8233352824615,21.3261189520454,-11.3142984672772));
#94647=CARTESIAN_POINT('Ctrl Pts',(18.8278002913827,21.3259256437256,-11.3145673944245));
#94648=CARTESIAN_POINT('Ctrl Pts',(18.8358238574311,21.3255528126936,-11.3150521583737));
#94649=CARTESIAN_POINT('Ctrl Pts',(18.8393825996404,21.3253784436563,-11.3152677038226));
#94650=CARTESIAN_POINT('Ctrl Pts',(18.8471261192545,21.3249794330817,-11.3157378880298));
#94651=CARTESIAN_POINT('Ctrl Pts',(18.8513106211726,21.3247513524082,-11.3159927119883));
#94652=CARTESIAN_POINT('Ctrl Pts',(18.8630926175503,21.3240740687784,-11.3167122389516));
#94653=CARTESIAN_POINT('Ctrl Pts',(18.8706883165142,21.3235963230442,-11.3171784956036));
#94654=CARTESIAN_POINT('Ctrl Pts',(18.9167068270839,21.320452687094,-11.3200171058944));
#94655=CARTESIAN_POINT('Ctrl Pts',(18.9550510197204,21.3167797699134,-11.3224405678));
#94656=CARTESIAN_POINT('Ctrl Pts',(19.0823648430219,21.3010692722043,-11.3306354298562));
#94657=CARTESIAN_POINT('Ctrl Pts',(19.1706640183234,21.2844199232623,-11.3365579453396));
#94658=CARTESIAN_POINT('Ctrl Pts',(19.4238479021482,21.219787298917,-11.3538250265188));
#94659=CARTESIAN_POINT('Ctrl Pts',(19.5843218646416,21.1573019400146,-11.3650715601222));
#94660=CARTESIAN_POINT('Ctrl Pts',(19.7560026546548,21.0651144753561,-11.3770690621102));
#94661=CARTESIAN_POINT('Ctrl Pts',(19.7763109033676,21.0537745283356,-11.3784890982728));
#94662=CARTESIAN_POINT('Ctrl Pts',(19.8047237576558,21.0372890253844,-11.3804777561737));
#94663=CARTESIAN_POINT('Ctrl Pts',(19.8129860064507,21.0324198231231,-11.3810562797581));
#94664=CARTESIAN_POINT('Ctrl Pts',(19.8263416651968,21.024426145331,-11.3819919138221));
#94665=CARTESIAN_POINT('Ctrl Pts',(19.8314553672487,21.0213359953691,-11.3823502684009));
#94666=CARTESIAN_POINT('Ctrl Pts',(19.8421199202348,21.0148297376691,-11.3830978784549));
#94667=CARTESIAN_POINT('Ctrl Pts',(19.8476682224185,21.0114095567289,-11.3834869795186));
#94668=CARTESIAN_POINT('Ctrl Pts',(19.8608077636216,21.0032258728076,-11.3844088635331));
#94669=CARTESIAN_POINT('Ctrl Pts',(19.8683847630615,20.9984396572793,-11.3849408017873));
#94670=CARTESIAN_POINT('Ctrl Pts',(19.8937060804997,20.9822189036811,-11.3867197736012));
#94671=CARTESIAN_POINT('Ctrl Pts',(19.9113100788448,20.9705668852392,-11.3879587104262));
#94672=CARTESIAN_POINT('Ctrl Pts',(20.0055409993628,20.9061483842077,-11.3946073244253));
#94673=CARTESIAN_POINT('Ctrl Pts',(20.078804807354,20.8486347238049,-11.3998314008981));
#94674=CARTESIAN_POINT('Ctrl Pts',(20.2632259593262,20.683109805168,-11.4134782156319));
#94675=CARTESIAN_POINT('Ctrl Pts',(20.3667062475343,20.5674303073793,-11.4216619975953));
#94676=CARTESIAN_POINT('Ctrl Pts',(20.4878082271995,20.3978948919597,-11.4333763599681));
#94677=CARTESIAN_POINT('Ctrl Pts',(20.5172970523708,20.3531091772455,-11.4364518106027));
#94678=CARTESIAN_POINT('Ctrl Pts',(20.549577226751,20.2997812907847,-11.4401509216324));
#94679=CARTESIAN_POINT('Ctrl Pts',(20.5540560298866,20.2922776736705,-11.4406722443179));
#94680=CARTESIAN_POINT('Ctrl Pts',(20.560764084092,20.2808794867444,-11.4414657359611));
#94681=CARTESIAN_POINT('Ctrl Pts',(20.5630276825952,20.277005098737,-11.44173572967));
#94682=CARTESIAN_POINT('Ctrl Pts',(20.5670671435151,20.2700403916653,-11.442221625785));
#94683=CARTESIAN_POINT('Ctrl Pts',(20.5688475333894,20.2669527606548,-11.4424372307562));
#94684=CARTESIAN_POINT('Ctrl Pts',(20.5726974245113,20.2602369736901,-11.4429066194741));
#94685=CARTESIAN_POINT('Ctrl Pts',(20.5747639609768,20.2566072327294,-11.4431605833631));
#94686=CARTESIAN_POINT('Ctrl Pts',(20.5805341218841,20.2464021868462,-11.44387530714));
#94687=CARTESIAN_POINT('Ctrl Pts',(20.5842133049146,20.2398132358139,-11.4443375883397));
#94688=CARTESIAN_POINT('Ctrl Pts',(20.6059098000369,20.2004647616597,-11.4471024736854));
#94689=CARTESIAN_POINT('Ctrl Pts',(20.6230907602157,20.1672544205329,-11.4494532142814));
#94690=CARTESIAN_POINT('Ctrl Pts',(20.6765544968016,20.056840541456,-11.4572826234238));
#94691=CARTESIAN_POINT('Ctrl Pts',(20.7090509171831,19.9779003835404,-11.4628991004263));
#94692=CARTESIAN_POINT('Ctrl Pts',(20.7943638057795,19.7289198915577,-11.4802860895096));
#94693=CARTESIAN_POINT('Ctrl Pts',(20.8305987731937,19.5539840016201,-11.4919767010469));
#94694=CARTESIAN_POINT('Ctrl Pts',(20.8462998904509,19.3538217910648,-11.5043325981684));
#94695=CARTESIAN_POINT('Ctrl Pts',(20.8477156735588,19.3310625102459,-11.5057243585255));
#94696=CARTESIAN_POINT('Ctrl Pts',(20.84920078048,19.298779221499,-11.5076805794816));
#94697=CARTESIAN_POINT('Ctrl Pts',(20.8495739469298,19.2892714070752,-11.5082545108053));
#94698=CARTESIAN_POINT('Ctrl Pts',(20.8500766254266,19.2738032695293,-11.5091847384302));
#94699=CARTESIAN_POINT('Ctrl Pts',(20.8502450821908,19.2678444242939,-11.5095422506322));
#94700=CARTESIAN_POINT('Ctrl Pts',(20.8505453138515,19.2553572855913,-11.5102897046013));
#94701=CARTESIAN_POINT('Ctrl Pts',(20.850672059687,19.2488289252443,-11.5106794849216));
#94702=CARTESIAN_POINT('Ctrl Pts',(20.8509020667678,19.2332739296784,-11.5116058889582));
#94703=CARTESIAN_POINT('Ctrl Pts',(20.8509778009979,19.2242469677634,-11.5121416453721));
#94704=CARTESIAN_POINT('Ctrl Pts',(20.8510386375244,19.1937256073128,-11.51394702882));
#94705=CARTESIAN_POINT('Ctrl Pts',(20.8507541321625,19.1722315662489,-11.5152082218536));
#94706=CARTESIAN_POINT('Ctrl Pts',(20.8450347463484,18.9713680465519,-11.5269079776311));
#94707=CARTESIAN_POINT('Ctrl Pts',(20.8171428806372,18.7933710984562,-11.536549798781));
#94708=CARTESIAN_POINT('Ctrl Pts',(20.7335446954159,18.5052876122127,-11.5528749525616));
#94709=CARTESIAN_POINT('Ctrl Pts',(20.6901482449709,18.392657448145,-11.5594858166961));
#94710=CARTESIAN_POINT('Ctrl Pts',(20.6332623359645,18.2758092422703,-11.5671880479486));
#94711=CARTESIAN_POINT('Ctrl Pts',(20.629048433378,18.2672995169497,-11.5677540744023));
#94712=CARTESIAN_POINT('Ctrl Pts',(20.6227172211405,18.2547274231828,-11.5685983089103));
#94713=CARTESIAN_POINT('Ctrl Pts',(20.6206436794066,18.2506429785462,-11.5688738452561));
#94714=CARTESIAN_POINT('Ctrl Pts',(20.6169297065753,18.2433856769471,-11.5693657251252));
#94715=CARTESIAN_POINT('Ctrl Pts',(20.6152944857216,18.24021021027,-11.5695817397259));
#94716=CARTESIAN_POINT('Ctrl Pts',(20.6117602214748,18.2333894206513,-11.5700474490644));
#94717=CARTESIAN_POINT('Ctrl Pts',(20.6098586237131,18.2297455389222,-11.5702972994488));
#94718=CARTESIAN_POINT('Ctrl Pts',(20.6045771761872,18.2196965768834,-11.5709891934025));
#94719=CARTESIAN_POINT('Ctrl Pts',(20.6011750893326,18.2133033371612,-11.5714326087916));
#94720=CARTESIAN_POINT('Ctrl Pts',(20.5823043108541,18.1782757462077,-11.5738792592153));
#94721=CARTESIAN_POINT('Ctrl Pts',(20.5662105856455,18.1499852449713,-11.5759188554206));
#94722=CARTESIAN_POINT('Ctrl Pts',(20.4657863631264,17.9825558733656,-11.5883250567758));
#94723=CARTESIAN_POINT('Ctrl Pts',(20.3662985886181,17.8531486721246,-11.5992814249176));
#94724=CARTESIAN_POINT('Ctrl Pts',(20.1716286397717,17.6526190376877,-11.6175367886597));
#94725=CARTESIAN_POINT('Ctrl Pts',(20.0834797711903,17.5756897918332,-11.6249758593466));
#94726=CARTESIAN_POINT('Ctrl Pts',(19.977903867916,17.4979335280801,-11.6329821446538));
#94727=CARTESIAN_POINT('Ctrl Pts',(19.9663015454054,17.4895684774626,-11.6338509484377));
#94728=CARTESIAN_POINT('Ctrl Pts',(19.9477042316927,17.4764445576263,-11.6352263157279));
#94729=CARTESIAN_POINT('Ctrl Pts',(19.9407641100374,17.4716090345565,-11.6357358143247));
#94730=CARTESIAN_POINT('Ctrl Pts',(19.9284749314416,17.4631555173197,-11.6366314693461));
#94731=CARTESIAN_POINT('Ctrl Pts',(19.9231379873602,17.4595201839791,-11.6370182831746));
#94732=CARTESIAN_POINT('Ctrl Pts',(19.9120669488827,17.4520529213889,-11.6378162993372));
#94733=CARTESIAN_POINT('Ctrl Pts',(19.9063305894001,17.4482244747865,-11.6382273669583));
#94734=CARTESIAN_POINT('Ctrl Pts',(19.8915620700298,17.4384719394702,-11.6392795606297));
#94735=CARTESIAN_POINT('Ctrl Pts',(19.88250302337,17.432588775566,-11.639919148345));
#94736=CARTESIAN_POINT('Ctrl Pts',(19.8445393624395,17.4083453262,-11.6425757237159));
#94737=CARTESIAN_POINT('Ctrl Pts',(19.8152355009437,17.3906177501525,-11.6445692748649));
#94738=CARTESIAN_POINT('Ctrl Pts',(19.7378064449826,17.3463062053433,-11.6497020610826));
#94739=CARTESIAN_POINT('Ctrl Pts',(19.689052331027,17.3208714294798,-11.6528021335327));
#94740=CARTESIAN_POINT('Ctrl Pts',(19.4687975385746,17.2166667699708,-11.6663520848232));
#94741=CARTESIAN_POINT('Ctrl Pts',(19.2882348186666,17.1591466038571,-11.676199034747));
#94742=CARTESIAN_POINT('Ctrl Pts',(19.0615060721991,17.1190729992212,-11.6892860808687));
#94743=CARTESIAN_POINT('Ctrl Pts',(19.0203485402759,17.1130431840534,-11.6916931939166));
#94744=CARTESIAN_POINT('Ctrl Pts',(18.9716773735515,17.107371358697,-11.6946045333284));
#94745=CARTESIAN_POINT('Ctrl Pts',(18.9643070613432,17.1065516997908,-11.6950471432882));
#94746=CARTESIAN_POINT('Ctrl Pts',(18.9523628739711,17.1052868730707,-11.6957674704168));
#94747=CARTESIAN_POINT('Ctrl Pts',(18.9477915162596,17.1048178368638,-11.6960438795591));
#94748=CARTESIAN_POINT('Ctrl Pts',(18.9396629405831,17.1040105545768,-11.6965367156421));
#94749=CARTESIAN_POINT('Ctrl Pts',(18.9361063568446,17.1036664268429,-11.6967528087136));
#94750=CARTESIAN_POINT('Ctrl Pts',(18.9284663623562,17.1029467158834,-11.6972180021051));
#94751=CARTESIAN_POINT('Ctrl Pts',(18.9243827872086,17.1025739974004,-11.6974672544637));
#94752=CARTESIAN_POINT('Ctrl Pts',(18.9131279491697,17.1015797024991,-11.6981558473679));
#94753=CARTESIAN_POINT('Ctrl Pts',(18.9059546370801,17.1009828405817,-11.698596538687));
#94754=CARTESIAN_POINT('Ctrl Pts',(18.8669668991856,17.0979389614568,-11.7010010834842));
#94755=CARTESIAN_POINT('Ctrl Pts',(18.8351051101092,17.0961750306914,-11.7029998679537));
#94756=CARTESIAN_POINT('Ctrl Pts',(18.6400669976789,17.0897946270919,-11.7153925853025));
#94757=CARTESIAN_POINT('Ctrl Pts',(18.4768512194941,17.1033449061866,-11.7263866650558));
#94758=CARTESIAN_POINT('Ctrl Pts',(18.2021472560211,17.1585620523851,-11.7446901786636));
#94759=CARTESIAN_POINT('Ctrl Pts',(18.0895729457072,17.1910766162971,-11.7521410671031));
#94760=CARTESIAN_POINT('Ctrl Pts',(17.9668806479234,17.2378245269314,-11.7601581549207));
#94761=CARTESIAN_POINT('Ctrl Pts',(17.9535675697509,17.2430521385401,-11.7610269113944));
#94762=CARTESIAN_POINT('Ctrl Pts',(17.9324669831045,17.2515854538265,-11.7624022181774));
#94763=CARTESIAN_POINT('Ctrl Pts',(17.9246447253978,17.2548035416535,-11.7629117031755));
#94764=CARTESIAN_POINT('Ctrl Pts',(17.9108849981836,17.2605609748596,-11.7638073423756));
#94765=CARTESIAN_POINT('Ctrl Pts',(17.9049395065154,17.2630807520377,-11.7641941539084));
#94766=CARTESIAN_POINT('Ctrl Pts',(17.8935303125682,17.2679778163649,-11.7649361045598));
#94767=CARTESIAN_POINT('Ctrl Pts',(17.8880649432119,17.2703510409135,-11.7652913774634));
#94768=CARTESIAN_POINT('Ctrl Pts',(17.8736608244107,17.2766781458925,-11.7662273665438));
#94769=CARTESIAN_POINT('Ctrl Pts',(17.8647392445906,17.2806709409273,-11.7668067473283));
#94770=CARTESIAN_POINT('Ctrl Pts',(17.8317010538587,17.2957324672595,-11.7689512898718));
#94771=CARTESIAN_POINT('Ctrl Pts',(17.8077649211115,17.3071928191867,-11.7705029649683));
#94772=CARTESIAN_POINT('Ctrl Pts',(17.7489473058214,17.3367259996946,-11.7743156033247));
#94773=CARTESIAN_POINT('Ctrl Pts',(17.7143408393757,17.3553256488277,-11.7765585052556));
#94774=CARTESIAN_POINT('Ctrl Pts',(17.5863822676452,17.4287596349442,-11.7848823970765));
#94775=CARTESIAN_POINT('Ctrl Pts',(17.4967606761279,17.4897655030613,-11.7907660869569));
#94776=CARTESIAN_POINT('Ctrl Pts',(17.3058049039953,17.6424022672289,-11.8040416132686));
#94777=CARTESIAN_POINT('Ctrl Pts',(17.2078836658889,17.7375011907802,-11.8113988810374));
#94778=CARTESIAN_POINT('Ctrl Pts',(17.1096883072435,17.8532282409597,-11.8202986671002));
#94779=CARTESIAN_POINT('Ctrl Pts',(17.0997220691599,17.8652406464747,-11.8212220557389));
#94780=CARTESIAN_POINT('Ctrl Pts',(17.0862500246481,17.881848991758,-11.8224999145189));
#94781=CARTESIAN_POINT('Ctrl Pts',(17.0826285856442,17.8863510525239,-11.8228464237323));
#94782=CARTESIAN_POINT('Ctrl Pts',(17.0769000683556,17.8935325675376,-11.8233994497365));
#94783=CARTESIAN_POINT('Ctrl Pts',(17.0747809227125,17.896202421572,-11.8236051096339));
#94784=CARTESIAN_POINT('Ctrl Pts',(17.0704149017352,17.9017304179976,-11.824031090084));
#94785=CARTESIAN_POINT('Ctrl Pts',(17.0681689443317,17.904589225887,-11.8242514755533));
#94786=CARTESIAN_POINT('Ctrl Pts',(17.0628304824508,17.911420534078,-11.8247782891491));
#94787=CARTESIAN_POINT('Ctrl Pts',(17.0597447723599,17.9153982957134,-11.8250851940471));
#94788=CARTESIAN_POINT('Ctrl Pts',(17.049365876394,17.9288766354773,-11.8261255129335));
#94789=CARTESIAN_POINT('Ctrl Pts',(17.0421392928358,17.9384278862813,-11.8268633810667));
#94790=CARTESIAN_POINT('Ctrl Pts',(16.9597880216623,18.0492114749439,-11.8354243973394));
#94791=CARTESIAN_POINT('Ctrl Pts',(16.8937765996098,18.1568880964307,-11.8437552150637));
#94792=CARTESIAN_POINT('Ctrl Pts',(16.8040373419541,18.3376845881892,-11.8570939358174));
#94793=CARTESIAN_POINT('Ctrl Pts',(16.7740037944131,18.4073511308399,-11.8620971063111));
#94794=CARTESIAN_POINT('Ctrl Pts',(16.7469837870813,18.4806160275211,-11.8671696042913));
#94795=CARTESIAN_POINT('Ctrl Pts',(16.7461998925523,18.4827521642303,-11.8673173404412));
#94796=CARTESIAN_POINT('Ctrl Pts',(16.745419450367,18.4848895417216,-11.8674650022761));
#94797=CARTESIAN_POINT('Ctrl Pts',(16.7454194497538,18.4848895434008,-11.642549296791));
#94798=CARTESIAN_POINT('Ctrl Pts',(16.7537303157283,18.4621287825794,-11.6410530257533));
#94799=CARTESIAN_POINT('Ctrl Pts',(16.7624319238914,18.4395107822216,-11.6395695084242));
#94800=CARTESIAN_POINT('Ctrl Pts',(16.775684223823,18.4067540355932,-11.6374251889696));
#94801=CARTESIAN_POINT('Ctrl Pts',(16.7799287754304,18.3964952994903,-11.636754235569));
#94802=CARTESIAN_POINT('Ctrl Pts',(16.7869663593863,18.3798577254545,-11.6356669465138));
#94803=CARTESIAN_POINT('Ctrl Pts',(16.7897104679755,18.3734585409185,-11.6352489590199));
#94804=CARTESIAN_POINT('Ctrl Pts',(16.7950506416844,18.3611730935298,-11.6344468462473));
#94805=CARTESIAN_POINT('Ctrl Pts',(16.7976420614972,18.3552849069457,-11.6340625679936));
#94806=CARTESIAN_POINT('Ctrl Pts',(16.8036402809634,18.3418226152657,-11.63318430541));
#94807=CARTESIAN_POINT('Ctrl Pts',(16.8070649042254,18.334256530857,-11.6326909381855));
#94808=CARTESIAN_POINT('Ctrl Pts',(16.8162885431216,18.3141936893783,-11.6313831862252));
#94809=CARTESIAN_POINT('Ctrl Pts',(16.82216522995,18.3017329237105,-11.6305714802213));
#94810=CARTESIAN_POINT('Ctrl Pts',(16.8683721768321,18.2061858018263,-11.6243495950424));
#94811=CARTESIAN_POINT('Ctrl Pts',(16.9139813992593,18.1257562142081,-11.619130978086));
#94812=CARTESIAN_POINT('Ctrl Pts',(17.041917556151,17.9310313317199,-11.6062461808229));
#94813=CARTESIAN_POINT('Ctrl Pts',(17.1306448023584,17.8214991450386,-11.5987713230542));
#94814=CARTESIAN_POINT('Ctrl Pts',(17.2668063055862,17.6839661268175,-11.588061457965));
#94815=CARTESIAN_POINT('Ctrl Pts',(17.3054348652333,17.6477691538067,-11.5850901223378));
#94816=CARTESIAN_POINT('Ctrl Pts',(17.3592463171664,17.6010065272359,-11.5809739587186));
#94817=CARTESIAN_POINT('Ctrl Pts',(17.3732725095626,17.5891346168386,-11.5799030318111));
#94818=CARTESIAN_POINT('Ctrl Pts',(17.3942177790491,17.571869284245,-11.5783036650403));
#94819=CARTESIAN_POINT('Ctrl Pts',(17.4010190524951,17.5663335624578,-11.5777843004343));
#94820=CARTESIAN_POINT('Ctrl Pts',(17.4133338152716,17.5564368420864,-11.5768434634185));
#94821=CARTESIAN_POINT('Ctrl Pts',(17.4188350463919,17.5520607133902,-11.5764230156726));
#94822=CARTESIAN_POINT('Ctrl Pts',(17.4275540980235,17.5451954933169,-11.575756204837));
#94823=CARTESIAN_POINT('Ctrl Pts',(17.4307575301666,17.5426880946719,-11.5755111232871));
#94824=CARTESIAN_POINT('Ctrl Pts',(17.4339774662751,17.5401827113813,-11.5752646653457));
#94825=CARTESIAN_POINT('Ctrl Pts',(17.4339867942605,17.5401754535432,-11.5752639513691));
#94826=CARTESIAN_POINT('Ctrl Pts',(17.4340054865226,17.5401609098811,-11.5752625206361));
#94827=CARTESIAN_POINT('Ctrl Pts',(17.434014850249,17.5401536244862,-11.5752618039219));
#94828=CARTESIAN_POINT('Ctrl Pts',(17.434033613905,17.5401390257819,-11.5752603677205));
#94829=CARTESIAN_POINT('Ctrl Pts',(17.43404301422,17.5401317121737,-11.5752596482038));
#94830=CARTESIAN_POINT('Ctrl Pts',(17.4340618514356,17.5401170567482,-11.5752582063681));
#94831=CARTESIAN_POINT('Ctrl Pts',(17.4340712881365,17.5401097150872,-11.5752574840644));
#94832=CARTESIAN_POINT('Ctrl Pts',(17.4340908542789,17.540094493086,-11.5752559864312));
#94833=CARTESIAN_POINT('Ctrl Pts',(17.434100984293,17.5400866123199,-11.5752552110577));
#94834=CARTESIAN_POINT('Ctrl Pts',(17.4341214209354,17.5400707136867,-11.5752536467901));
#94835=CARTESIAN_POINT('Ctrl Pts',(17.4341317269927,17.5400626962691,-11.5752528579396));
#94836=CARTESIAN_POINT('Ctrl Pts',(17.434152519508,17.5400465214031,-11.575251266428));
#94837=CARTESIAN_POINT('Ctrl Pts',(17.4341630058967,17.540038364014,-11.5752504637721));
#94838=CARTESIAN_POINT('Ctrl Pts',(17.4341841625331,17.5400219065311,-11.5752488443848));
#94839=CARTESIAN_POINT('Ctrl Pts',(17.4341948330354,17.5400136062448,-11.5752480276338));
#94840=CARTESIAN_POINT('Ctrl Pts',(17.4342163619203,17.5399968598565,-11.5752463797486));
#94841=CARTESIAN_POINT('Ctrl Pts',(17.4342272202797,17.5399884137783,-11.5752455486159));
#94842=CARTESIAN_POINT('Ctrl Pts',(17.4342491291808,17.5399713724772,-11.5752438716378));
#94843=CARTESIAN_POINT('Ctrl Pts',(17.4342601794598,17.5399627774648,-11.5752430258124));
#94844=CARTESIAN_POINT('Ctrl Pts',(17.4342824761245,17.5399454352613,-11.5752413191482));
#94845=CARTESIAN_POINT('Ctrl Pts',(17.43429372272,17.5399366879134,-11.5752404582932));
#94846=CARTESIAN_POINT('Ctrl Pts',(17.4343164162529,17.5399190377637,-11.5752387212457));
#94847=CARTESIAN_POINT('Ctrl Pts',(17.4343278632199,17.5399101349456,-11.5752378450508));
#94848=CARTESIAN_POINT('Ctrl Pts',(17.4343509618229,17.5398921705099,-11.5752360769918));
#94849=CARTESIAN_POINT('Ctrl Pts',(17.4343626136718,17.5398831087336,-11.5752351851114));
#94850=CARTESIAN_POINT('Ctrl Pts',(17.434386126887,17.5398648226317,-11.5752333853103));
#94851=CARTESIAN_POINT('Ctrl Pts',(17.4343979878672,17.5398555986133,-11.5752324774191));
#94852=CARTESIAN_POINT('Ctrl Pts',(17.434421923896,17.5398369845094,-11.5752306452478));
#94853=CARTESIAN_POINT('Ctrl Pts',(17.434433998984,17.5398275944005,-11.5752297209646));
#94854=CARTESIAN_POINT('Ctrl Pts',(17.4344583676632,17.5398086446891,-11.5752278556698));
#94855=CARTESIAN_POINT('Ctrl Pts',(17.4344706615746,17.5397990848452,-11.5752269146336));
#94856=CARTESIAN_POINT('Ctrl Pts',(17.4344954730773,17.5397797916615,-11.5752250154361));
#94857=CARTESIAN_POINT('Ctrl Pts',(17.4345079904292,17.5397700585159,-11.5752240572932));
#94858=CARTESIAN_POINT('Ctrl Pts',(17.4345332538001,17.5397504148748,-11.5752221235005));
#94859=CARTESIAN_POINT('Ctrl Pts',(17.4345459999316,17.5397405043002,-11.575221147842));
#94860=CARTESIAN_POINT('Ctrl Pts',(17.437250611522,17.5376376213878,-11.5750141217284));
#94861=CARTESIAN_POINT('Ctrl Pts',(17.4399474717246,17.5355512003818,-11.5748076050558));
#94862=CARTESIAN_POINT('Ctrl Pts',(17.4462709869107,17.530683399605,-11.5743231848071));
#94863=CARTESIAN_POINT('Ctrl Pts',(17.4499016039276,17.5279072524029,-11.5740449174992));
#94864=CARTESIAN_POINT('Ctrl Pts',(17.4610616695905,17.5194308488903,-11.5731892055801));
#94865=CARTESIAN_POINT('Ctrl Pts',(17.468620175123,17.5137692916967,-11.5726091579254));
#94866=CARTESIAN_POINT('Ctrl Pts',(17.5754084836177,17.4348913575707,-11.5644102390713));
#94867=CARTESIAN_POINT('Ctrl Pts',(17.6808018981422,17.3704394858355,-11.5562848639047));
#94868=CARTESIAN_POINT('Ctrl Pts',(17.8857840624119,17.2684808440113,-11.5411575016869));
#94869=CARTESIAN_POINT('Ctrl Pts',(17.9837751780056,17.2285729770792,-11.5341809049508));
#94870=CARTESIAN_POINT('Ctrl Pts',(18.1555570656964,17.1731846035542,-11.5225856324242));
#94871=CARTESIAN_POINT('Ctrl Pts',(18.2279451053839,17.1540123016869,-11.5178784450629));
#94872=CARTESIAN_POINT('Ctrl Pts',(18.3195866473613,17.1348730200115,-11.5121434907082));
#94873=CARTESIAN_POINT('Ctrl Pts',(18.338020080335,17.1312784795129,-11.5110008996551));
#94874=CARTESIAN_POINT('Ctrl Pts',(18.3649114913913,17.126405132787,-11.5093495386187));
#94875=CARTESIAN_POINT('Ctrl Pts',(18.3733328529419,17.1249316166578,-11.5088345946421));
#94876=CARTESIAN_POINT('Ctrl Pts',(18.3881215259821,17.1224362200008,-11.5079340935157));
#94877=CARTESIAN_POINT('Ctrl Pts',(18.3944849675306,17.1213923511654,-11.5075478422133));
#94878=CARTESIAN_POINT('Ctrl Pts',(18.4068564931693,17.1194209119807,-11.5067992546602));
#94879=CARTESIAN_POINT('Ctrl Pts',(18.4128639921794,17.1184901144396,-11.5064368195371));
#94880=CARTESIAN_POINT('Ctrl Pts',(18.4272443835318,17.1163254148662,-11.5055717660214));
#94881=CARTESIAN_POINT('Ctrl Pts',(18.4356208709167,17.1151158132358,-11.5050699199557));
#94882=CARTESIAN_POINT('Ctrl Pts',(18.4659300130887,17.1109244288998,-11.5032612523006));
#94883=CARTESIAN_POINT('Ctrl Pts',(18.4879023268843,17.1082363632617,-11.5019636897966));
#94884=CARTESIAN_POINT('Ctrl Pts',(18.6941992808494,17.0862762480149,-11.4898979823811));
#94885=CARTESIAN_POINT('Ctrl Pts',(18.8802578409069,17.090941085481,-11.4799835944544));
#94886=CARTESIAN_POINT('Ctrl Pts',(19.1426782767497,17.1322693759548,-11.4655024263769));
#94887=CARTESIAN_POINT('Ctrl Pts',(19.2212307941875,17.1492669720571,-11.4610863327069));
#94888=CARTESIAN_POINT('Ctrl Pts',(19.3333901630184,17.1803050707585,-11.454429905064));
#94889=CARTESIAN_POINT('Ctrl Pts',(19.3679052646057,17.1908133183191,-11.4523315833809));
#94890=CARTESIAN_POINT('Ctrl Pts',(19.409219946611,17.2045546830729,-11.4497404917154));
#94891=CARTESIAN_POINT('Ctrl Pts',(19.4162945803703,17.2069493798944,-11.4492939543135));
#94892=CARTESIAN_POINT('Ctrl Pts',(19.4272894743913,17.210736015001,-11.4485953252124));
#94893=CARTESIAN_POINT('Ctrl Pts',(19.4312186348412,17.2121021838192,-11.4483447328549));
#94894=CARTESIAN_POINT('Ctrl Pts',(19.4385082998727,17.2146609078947,-11.4478780447719));
#94895=CARTESIAN_POINT('Ctrl Pts',(19.4418698272535,17.2158503759576,-11.4476621328499));
#94896=CARTESIAN_POINT('Ctrl Pts',(19.4494759398482,17.2185634220459,-11.4471719970456));
#94897=CARTESIAN_POINT('Ctrl Pts',(19.4537186499034,17.2200920659705,-11.4468974759139));
#94898=CARTESIAN_POINT('Ctrl Pts',(19.4646596249247,17.2240736308564,-11.4461867090372));
#94899=CARTESIAN_POINT('Ctrl Pts',(19.4713503717001,17.2265468486405,-11.4457492975838));
#94900=CARTESIAN_POINT('Ctrl Pts',(19.5123412425618,17.2419349410125,-11.4430531143187));
#94901=CARTESIAN_POINT('Ctrl Pts',(19.5463114948161,17.2557041250254,-11.4407481931253));
#94902=CARTESIAN_POINT('Ctrl Pts',(19.7361891263442,17.338469255174,-11.4275297172256));
#94903=CARTESIAN_POINT('Ctrl Pts',(19.8836712324236,17.4252190568367,-11.4160261126721));
#94904=CARTESIAN_POINT('Ctrl Pts',(20.0949859578043,17.5866501800109,-11.3987444948252));
#94905=CARTESIAN_POINT('Ctrl Pts',(20.1668205443087,17.6496465295991,-11.3926814966654));
#94906=CARTESIAN_POINT('Ctrl Pts',(20.2492640454183,17.7324460840374,-11.3855042061676));
#94907=CARTESIAN_POINT('Ctrl Pts',(20.2641306937055,17.7478366725905,-11.3842000039093));
#94908=CARTESIAN_POINT('Ctrl Pts',(20.2849231306298,17.7700254567663,-11.3823609872685));
#94909=CARTESIAN_POINT('Ctrl Pts',(20.2910423941322,17.7766398018038,-11.381817860106));
#94910=CARTESIAN_POINT('Ctrl Pts',(20.3015207911573,17.7881120337705,-11.3808844548083));
#94911=CARTESIAN_POINT('Ctrl Pts',(20.3058999963008,17.7929513413632,-11.380493325479));
#94912=CARTESIAN_POINT('Ctrl Pts',(20.3142383720796,17.8022518809185,-11.3797465565772));
#94913=CARTESIAN_POINT('Ctrl Pts',(20.3182011981886,17.8067097378434,-11.379390764956));
#94914=CARTESIAN_POINT('Ctrl Pts',(20.3284490254618,17.8183362952035,-11.3784683300911));
#94915=CARTESIAN_POINT('Ctrl Pts',(20.3347045810452,17.825530859891,-11.3779029180621));
#94916=CARTESIAN_POINT('Ctrl Pts',(20.355829665661,17.8501610583487,-11.375985266427));
#94917=CARTESIAN_POINT('Ctrl Pts',(20.3704649459568,17.8677961321829,-11.3746426438942));
#94918=CARTESIAN_POINT('Ctrl Pts',(20.4953050086257,18.0232945841486,-11.3630542855609));
#94919=CARTESIAN_POINT('Ctrl Pts',(20.5881539763528,18.1741976220399,-11.3535696039358));
#94920=CARTESIAN_POINT('Ctrl Pts',(20.6969165631051,18.413444741087,-11.3392675806512));
#94921=CARTESIAN_POINT('Ctrl Pts',(20.7277899346988,18.494107283399,-11.3345411645067));
#94922=CARTESIAN_POINT('Ctrl Pts',(20.7649367519452,18.612333223203,-11.3274644531751));
#94923=CARTESIAN_POINT('Ctrl Pts',(20.7752597745061,18.6485374331556,-11.3252775754328));
#94924=CARTESIAN_POINT('Ctrl Pts',(20.7864902979372,18.6923192200176,-11.3225882826959));
#94925=CARTESIAN_POINT('Ctrl Pts',(20.7883297695293,18.6996533770857,-11.3221362898946));
#94926=CARTESIAN_POINT('Ctrl Pts',(20.7911250362954,18.7110569455564,-11.3214309675287));
#94927=CARTESIAN_POINT('Ctrl Pts',(20.7921081565871,18.7151196840608,-11.3211791841287));
#94928=CARTESIAN_POINT('Ctrl Pts',(20.7939072000034,18.7226517335949,-11.3207114257733));
#94929=CARTESIAN_POINT('Ctrl Pts',(20.7947263971961,18.7261202033062,-11.320495641889));
#94930=CARTESIAN_POINT('Ctrl Pts',(20.7965562803961,18.7339563041672,-11.3200072733806));
#94931=CARTESIAN_POINT('Ctrl Pts',(20.7975618477738,18.7383250619169,-11.3197344006999));
#94932=CARTESIAN_POINT('Ctrl Pts',(20.8004823201187,18.7512002102937,-11.318928523378));
#94933=CARTESIAN_POINT('Ctrl Pts',(20.8023585299626,18.7597151548073,-11.318393382518));
#94934=CARTESIAN_POINT('Ctrl Pts',(20.8153373852477,18.8203996581062,-11.3145652512978));
#94935=CARTESIAN_POINT('Ctrl Pts',(20.8245165545187,18.8729564556639,-11.3111752227075));
#94936=CARTESIAN_POINT('Ctrl Pts',(20.834092808793,18.9433912930584,-11.3065812275964));
#94937=CARTESIAN_POINT('Ctrl Pts',(20.8362632431785,18.9610130860804,-11.3054276363247));
#94938=CARTESIAN_POINT('Ctrl Pts',(20.8435209819836,19.0267434879935,-11.301113365274));
#94939=CARTESIAN_POINT('Ctrl Pts',(20.8471803864982,19.074993919207,-11.2979242541586));
#94940=CARTESIAN_POINT('Ctrl Pts',(20.8537136925562,19.232613474925,-11.287503402309));
#94941=CARTESIAN_POINT('Ctrl Pts',(20.8497671240275,19.3420962371424,-11.2802707081327));
#94942=CARTESIAN_POINT('Ctrl Pts',(20.8311348064382,19.50553451864,-11.2696972801468));
#94943=CARTESIAN_POINT('Ctrl Pts',(20.8227584661425,19.5600184381416,-11.2662081684419));
#94944=CARTESIAN_POINT('Ctrl Pts',(20.8057330654138,19.647792627328,-11.2606506343006));
#94945=CARTESIAN_POINT('Ctrl Pts',(20.7983833242257,19.6813056459291,-11.2585437737274));
#94946=CARTESIAN_POINT('Ctrl Pts',(20.7876507349811,19.7251249658662,-11.2558072506868));
#94947=CARTESIAN_POINT('Ctrl Pts',(20.7849990549321,19.7356033790098,-11.2551542470154));
#94948=CARTESIAN_POINT('Ctrl Pts',(20.780523766397,19.7527352268918,-11.2540887483289));
#94949=CARTESIAN_POINT('Ctrl Pts',(20.7787477045698,19.7594007739709,-11.2536747238756));
#94950=CARTESIAN_POINT('Ctrl Pts',(20.7752461823634,19.7722884396261,-11.252875208879));
#94951=CARTESIAN_POINT('Ctrl Pts',(20.7735247749198,19.7785115711466,-11.2524895919934));
#94952=CARTESIAN_POINT('Ctrl Pts',(20.7694836224523,19.7928650218427,-11.2516011714039));
#94953=CARTESIAN_POINT('Ctrl Pts',(20.7671435796942,19.800989549422,-11.2510990337664));
#94954=CARTESIAN_POINT('Ctrl Pts',(20.7607177169652,19.8228075626819,-11.2497524230434));
#94955=CARTESIAN_POINT('Ctrl Pts',(20.7565417741932,19.8364742077569,-11.2489108913707));
#94956=CARTESIAN_POINT('Ctrl Pts',(20.716956134961,19.9614829877329,-11.2412290520041));
#94957=CARTESIAN_POINT('Ctrl Pts',(20.6725224675458,20.0697640270365,-11.2347054284596));
#94958=CARTESIAN_POINT('Ctrl Pts',(20.5453373570925,20.3188107702178,-11.2193964995653));
#94959=CARTESIAN_POINT('Ctrl Pts',(20.4548364695359,20.4547434210946,-11.2107943962046));
#94960=CARTESIAN_POINT('Ctrl Pts',(20.3286974594612,20.6037249329809,-11.1995852224268));
#94961=CARTESIAN_POINT('Ctrl Pts',(20.307156146158,20.6280117168745,-11.1976918670049));
#94962=CARTESIAN_POINT('Ctrl Pts',(20.2801414461308,20.657094047366,-11.1953284605241));
#94963=CARTESIAN_POINT('Ctrl Pts',(20.2751894210102,20.6623705696336,-11.1948956644689));
#94964=CARTESIAN_POINT('Ctrl Pts',(20.2673832948863,20.6706032182577,-11.1942139092523));
#94965=CARTESIAN_POINT('Ctrl Pts',(20.264547419957,20.6735766572689,-11.1939663342924));
#94966=CARTESIAN_POINT('Ctrl Pts',(20.2592301031966,20.6791195086974,-11.1935022677287));
#94967=CARTESIAN_POINT('Ctrl Pts',(20.2567508088608,20.6816909032737,-11.1932859412293));
#94968=CARTESIAN_POINT('Ctrl Pts',(20.2510759262806,20.6875468614301,-11.192790918483));
#94969=CARTESIAN_POINT('Ctrl Pts',(20.2478761845755,20.690827319981,-11.192511899994));
#94970=CARTESIAN_POINT('Ctrl Pts',(20.2380064594572,20.7008805082811,-11.1916516277518));
#94971=CARTESIAN_POINT('Ctrl Pts',(20.2313015975227,20.7076186145295,-11.1910677312704));
#94972=CARTESIAN_POINT('Ctrl Pts',(20.1699489746241,20.7684505026365,-11.1857314418229));
#94973=CARTESIAN_POINT('Ctrl Pts',(20.1124428459899,20.8195689972922,-11.180778892149));
#94974=CARTESIAN_POINT('Ctrl Pts',(19.9424160350423,20.9548861742614,-11.1665611288904));
#94975=CARTESIAN_POINT('Ctrl Pts',(19.8241015915385,21.0311899909556,-11.1571727597118));
#94976=CARTESIAN_POINT('Ctrl Pts',(19.643972914943,21.1234525820152,-11.1440958692517));
#94977=CARTESIAN_POINT('Ctrl Pts',(19.5876273275295,21.1492587823443,-11.1401556591136));
#94978=CARTESIAN_POINT('Ctrl Pts',(19.4956516973328,21.1865930970191,-11.1339701548899));
#94979=CARTESIAN_POINT('Ctrl Pts',(19.4607101614286,21.1997116463354,-11.1316747066117));
#94980=CARTESIAN_POINT('Ctrl Pts',(19.4149083637398,21.2155390790436,-11.1287338360591));
#94981=CARTESIAN_POINT('Ctrl Pts',(19.4043497533942,21.2190947026425,-11.128060492888));
#94982=CARTESIAN_POINT('Ctrl Pts',(19.3871393373693,21.2247394579314,-11.1269703016982));
#94983=CARTESIAN_POINT('Ctrl Pts',(19.3805045170662,21.2268793390655,-11.1265517852828));
#94984=CARTESIAN_POINT('Ctrl Pts',(19.3677296186385,21.2309299788452,-11.1257493054663));
#94985=CARTESIAN_POINT('Ctrl Pts',(19.361591177199,21.2328456085191,-11.1253651856213));
#94986=CARTESIAN_POINT('Ctrl Pts',(19.3475229199278,21.2371656614455,-11.1244881821812));
#94987=CARTESIAN_POINT('Ctrl Pts',(19.3395874926901,21.2395515651752,-11.1239959096082));
#94988=CARTESIAN_POINT('Ctrl Pts',(19.318483101908,21.2457620366185,-11.1226929811458));
#94989=CARTESIAN_POINT('Ctrl Pts',(19.3052905030726,21.2495053878711,-11.1218849722252));
#94990=CARTESIAN_POINT('Ctrl Pts',(19.2053492726639,21.2768169150562,-11.1158107534666));
#94991=CARTESIAN_POINT('Ctrl Pts',(19.1172093912315,21.2949681044395,-11.110725416215));
#94992=CARTESIAN_POINT('Ctrl Pts',(18.8901023292052,21.3268355391554,-11.0980275873393));
#94993=CARTESIAN_POINT('Ctrl Pts',(18.7504613617129,21.3325219043984,-11.090611099825));
#94994=CARTESIAN_POINT('Ctrl Pts',(18.5557493997068,21.3212155361911,-11.0798403700041));
#94995=CARTESIAN_POINT('Ctrl Pts',(18.5003726130913,21.3158040923634,-11.0767245883081));
#94996=CARTESIAN_POINT('Ctrl Pts',(18.4169477110041,21.3043190448105,-11.0718677501062));
#94997=CARTESIAN_POINT('Ctrl Pts',(18.3887016049855,21.2998455217526,-11.0701946530488));
#94998=CARTESIAN_POINT('Ctrl Pts',(18.3537129044125,21.2935751036294,-11.0680768213649));
#94999=CARTESIAN_POINT('Ctrl Pts',(18.3468756188353,21.2923149804333,-11.0676608022763));
#95000=CARTESIAN_POINT('Ctrl Pts',(18.3360691591824,21.2902682410911,-11.0669996716658));
#95001=CARTESIAN_POINT('Ctrl Pts',(18.3320957506295,21.2895038720654,-11.0667558091685));
#95002=CARTESIAN_POINT('Ctrl Pts',(18.3246080495659,21.2880411813226,-11.0662947629143));
#95003=CARTESIAN_POINT('Ctrl Pts',(18.321093329879,21.2873453275034,-11.0660777205625));
#95004=CARTESIAN_POINT('Ctrl Pts',(18.3130642432425,21.2857345144377,-11.0655804829601));
#95005=CARTESIAN_POINT('Ctrl Pts',(18.3085510904496,21.28481374312,-11.0652999594098));
#95006=CARTESIAN_POINT('Ctrl Pts',(18.2965825301838,21.28233120955,-11.0645533721343));
#95007=CARTESIAN_POINT('Ctrl Pts',(18.2891325644589,21.2807439414929,-11.0640859085787));
#95008=CARTESIAN_POINT('Ctrl Pts',(18.2371681829844,21.2693790433653,-11.0608069054905));
#95009=CARTESIAN_POINT('Ctrl Pts',(18.1929744732382,21.2582070830349,-11.0579240295177));
#95010=CARTESIAN_POINT('Ctrl Pts',(18.1432661850623,21.2439191858732,-11.0545994519143));
#95011=CARTESIAN_POINT('Ctrl Pts',(18.1373603453429,21.2421937321747,-11.0542031267414));
#95012=CARTESIAN_POINT('Ctrl Pts',(18.1271215696667,21.2391538581471,-11.0535138048808));
#95013=CARTESIAN_POINT('Ctrl Pts',(18.1227851482519,21.2378512293834,-11.0532211618298));
#95014=CARTESIAN_POINT('Ctrl Pts',(18.0946964125259,21.2293152423388,-11.051321217674));
#95015=CARTESIAN_POINT('Ctrl Pts',(18.0710692840745,21.2216785667851,-11.0497027582124));
#95016=CARTESIAN_POINT('Ctrl Pts',(18.0104645888448,21.2009058054057,-11.0455069403706));
#95017=CARTESIAN_POINT('Ctrl Pts',(17.9737081440305,21.1871540401087,-11.0429190833576));
#95018=CARTESIAN_POINT('Ctrl Pts',(17.8360959829326,21.1312610353945,-11.033107423052));
#95019=CARTESIAN_POINT('Ctrl Pts',(17.73816525062,21.0823499640679,-11.0258810809025));
#95020=CARTESIAN_POINT('Ctrl Pts',(17.5972933620927,20.9977880025836,-11.0153209921847));
#95021=CARTESIAN_POINT('Ctrl Pts',(17.5512600005505,20.9676559871331,-11.011838823645));
#95022=CARTESIAN_POINT('Ctrl Pts',(17.4785407936619,20.9159001720591,-11.0062910547081));
#95023=CARTESIAN_POINT('Ctrl Pts',(17.4511174496957,20.8953618949057,-11.004187184367));
#95024=CARTESIAN_POINT('Ctrl Pts',(17.4157162759546,20.867482334929,-11.0014539183714));
#95025=CARTESIAN_POINT('Ctrl Pts',(17.4072804091997,20.8607335655119,-11.000801250945));
#95026=CARTESIAN_POINT('Ctrl Pts',(17.3935441125473,20.8495708955155,-10.9997361602729));
#95027=CARTESIAN_POINT('Ctrl Pts',(17.3882130165235,20.8451952033627,-10.9993222098493));
#95028=CARTESIAN_POINT('Ctrl Pts',(17.3779321895364,20.8366724114031,-10.9985227406241));
#95029=CARTESIAN_POINT('Ctrl Pts',(17.3729798688147,20.832528568884,-10.9981370959896));
#95030=CARTESIAN_POINT('Ctrl Pts',(17.3615850302393,20.8229049854075,-10.9972484725364));
#95031=CARTESIAN_POINT('Ctrl Pts',(17.3551562083799,20.8174091423676,-10.9967461607605));
#95032=CARTESIAN_POINT('Ctrl Pts',(17.3379467302571,20.8025177534045,-10.9953987745792));
#95033=CARTESIAN_POINT('Ctrl Pts',(17.3272279334716,20.7930511556645,-10.9945566469522));
#95034=CARTESIAN_POINT('Ctrl Pts',(17.2292160350151,20.7047054740705,-10.9868265727809));
#95035=CARTESIAN_POINT('Ctrl Pts',(17.1485393427668,20.6187821816334,-10.9802600960631));
#95036=CARTESIAN_POINT('Ctrl Pts',(16.9737389830966,20.3984080756374,-10.9648655756459));
#95037=CARTESIAN_POINT('Ctrl Pts',(16.8872806450838,20.2588893352109,-10.9562204814614));
#95038=CARTESIAN_POINT('Ctrl Pts',(16.8045807840989,20.0827747064493,-10.9450299597384));
#95039=CARTESIAN_POINT('Ctrl Pts',(16.7920251373158,20.0544352694506,-10.9432200695927));
#95040=CARTESIAN_POINT('Ctrl Pts',(16.7773512455881,20.0192484369357,-10.9409495898788));
#95041=CARTESIAN_POINT('Ctrl Pts',(16.7746389808925,20.0126509698459,-10.9405228850975));
#95042=CARTESIAN_POINT('Ctrl Pts',(16.7704255502863,20.0022528534787,-10.9398486156054));
#95043=CARTESIAN_POINT('Ctrl Pts',(16.7689019287751,19.9984612800167,-10.939602385333));
#95044=CARTESIAN_POINT('Ctrl Pts',(16.7660657187978,19.9913438021033,-10.9391394410906));
#95045=CARTESIAN_POINT('Ctrl Pts',(16.7647505755529,19.9880189754749,-10.938922883739));
#95046=CARTESIAN_POINT('Ctrl Pts',(16.7617562475997,19.9803925555127,-10.9384254733093));
#95047=CARTESIAN_POINT('Ctrl Pts',(16.7600827149697,19.976088801569,-10.9381442859707));
#95048=CARTESIAN_POINT('Ctrl Pts',(16.7549425689509,19.9627409778176,-10.9372707693427));
#95049=CARTESIAN_POINT('Ctrl Pts',(16.7515239901557,19.9536787160888,-10.9366756803647));
#95050=CARTESIAN_POINT('Ctrl Pts',(16.7114754925612,19.845267729969,-10.9295352472));
#95051=CARTESIAN_POINT('Ctrl Pts',(16.6822910932671,19.7433402800352,-10.9226144786129));
#95052=CARTESIAN_POINT('Ctrl Pts',(16.6317924910195,19.4991187845646,-10.9061647804671));
#95053=CARTESIAN_POINT('Ctrl Pts',(16.6170952312495,19.3559559289461,-10.8966461787978));
#95054=CARTESIAN_POINT('Ctrl Pts',(16.616959535722,19.1504033908249,-10.8835935562426));
#95055=CARTESIAN_POINT('Ctrl Pts',(16.6196417426167,19.08843294355,-10.8797325138413));
#95056=CARTESIAN_POINT('Ctrl Pts',(16.626121996496,19.0142932853695,-10.875199725925));
#95057=CARTESIAN_POINT('Ctrl Pts',(16.6273121374375,19.0019319027675,-10.8744468144049));
#95058=CARTESIAN_POINT('Ctrl Pts',(16.6294460867381,18.9816409454271,-10.8732154433114));
#95059=CARTESIAN_POINT('Ctrl Pts',(16.630326098969,18.9737050978484,-10.8727349879567));
#95060=CARTESIAN_POINT('Ctrl Pts',(16.631989697049,18.959440158749,-10.8718733437355));
#95061=CARTESIAN_POINT('Ctrl Pts',(16.6327570210524,18.9531093017493,-10.8714916473455));
#95062=CARTESIAN_POINT('Ctrl Pts',(16.6344530082319,18.9396267583189,-10.8706802318216));
#95063=CARTESIAN_POINT('Ctrl Pts',(16.635389633832,18.9324761411828,-10.8702507690383));
#95064=CARTESIAN_POINT('Ctrl Pts',(16.6380125543847,18.9132163550913,-10.869096331034));
#95065=CARTESIAN_POINT('Ctrl Pts',(16.6397672532844,18.9011166616507,-10.8683735224932));
#95066=CARTESIAN_POINT('Ctrl Pts',(16.6490971359134,18.8404844345048,-10.8647629891558));
#95067=CARTESIAN_POINT('Ctrl Pts',(16.6582553257513,18.7922084812765,-10.8619257832645));
#95068=CARTESIAN_POINT('Ctrl Pts',(16.6889757434457,18.656288321238,-10.8540036612939));
#95069=CARTESIAN_POINT('Ctrl Pts',(16.7144720714676,18.5696443543303,-10.8490363878053));
#95070=CARTESIAN_POINT('Ctrl Pts',(16.7454194500511,18.4848895425866,-10.8441190257052));
#95071=CARTESIAN_POINT('Origin',(18.734,19.211,0.));
#95072=CARTESIAN_POINT('',(16.7454194503153,18.4848895418633,-10.0464611586511));
#95073=CARTESIAN_POINT('',(16.7460269850049,18.48512090247,-10.2662522550585));
#95074=CARTESIAN_POINT('',(16.7454194503191,18.4848895418526,0.));
#95075=CARTESIAN_POINT('',(16.6141769831468,19.2099225630115,-10.3109437209775));
#95076=CARTESIAN_POINT('Ctrl Pts',(16.746026985005,18.4851209024697,-10.2662522550585));
#95077=CARTESIAN_POINT('Ctrl Pts',(16.6804601501866,18.6593671879511,-10.2774434318084));
#95078=CARTESIAN_POINT('Ctrl Pts',(16.6235837846056,18.9018894313097,-10.2923405871147));
#95079=CARTESIAN_POINT('Ctrl Pts',(16.6137958787386,19.1485339243464,-10.307237742421));
#95080=CARTESIAN_POINT('Ctrl Pts',(16.6141769831468,19.2099225630115,-10.3109437209775));
#95081=CARTESIAN_POINT('Ctrl Pts',(16.6170002227485,19.2100288578692,-10.3093226092216));
#95082=CARTESIAN_POINT('Ctrl Pts',(16.6169204631466,19.3838973927067,-10.3205065096121));
#95083=CARTESIAN_POINT('Ctrl Pts',(16.6382591297735,19.5571243916928,-10.3322373725637));
#95084=CARTESIAN_POINT('Ctrl Pts',(16.6953904168952,19.7850075989709,-10.3474076082501));
#95085=CARTESIAN_POINT('Ctrl Pts',(16.7127857427009,19.8435407289489,-10.3512876713133));
#95086=CARTESIAN_POINT('Ctrl Pts',(16.7447265731386,19.9361507375324,-10.3573901651957));
#95087=CARTESIAN_POINT('Ctrl Pts',(16.7576771892852,19.9707373073503,-10.3596610984453));
#95088=CARTESIAN_POINT('Ctrl Pts',(16.7756892746449,20.0152582265561,-10.3625755207103));
#95089=CARTESIAN_POINT('Ctrl Pts',(16.7799328772434,20.0255145051719,-10.3632463129835));
#95090=CARTESIAN_POINT('Ctrl Pts',(16.7869692717986,20.0421490922638,-10.3643334064241));
#95091=CARTESIAN_POINT('Ctrl Pts',(16.7897131730314,20.0485477338096,-10.3647513583161));
#95092=CARTESIAN_POINT('Ctrl Pts',(16.7950532285592,20.0608328100748,-10.3655534466433));
#95093=CARTESIAN_POINT('Ctrl Pts',(16.7976447444331,20.0667211655728,-10.3659377358185));
#95094=CARTESIAN_POINT('Ctrl Pts',(16.803643604065,20.0801847771502,-10.3668160842831));
#95095=CARTESIAN_POINT('Ctrl Pts',(16.8070687834751,20.0877520070919,-10.3673095260527));
#95096=CARTESIAN_POINT('Ctrl Pts',(16.8162948647742,20.1078198951483,-10.3686176065359));
#95097=CARTESIAN_POINT('Ctrl Pts',(16.8221735008295,20.1202845321845,-10.3694295643482));
#95098=CARTESIAN_POINT('Ctrl Pts',(16.8684550180522,20.2159831237312,-10.3756613105747));
#95099=CARTESIAN_POINT('Ctrl Pts',(16.9141559267543,20.2965504389374,-10.3808888114111));
#95100=CARTESIAN_POINT('Ctrl Pts',(17.0421916993997,20.4913233443882,-10.3937778197207));
#95101=CARTESIAN_POINT('Ctrl Pts',(17.1308960704148,20.6007836880026,-10.4012490349878));
#95102=CARTESIAN_POINT('Ctrl Pts',(17.2669770060914,20.7381953313056,-10.4119516171495));
#95103=CARTESIAN_POINT('Ctrl Pts',(17.3055554878535,20.774338593815,-10.4149190303441));
#95104=CARTESIAN_POINT('Ctrl Pts',(17.3593008957968,20.8210398823636,-10.419030117648));
#95105=CARTESIAN_POINT('Ctrl Pts',(17.3733145398385,20.8329004538023,-10.4201000852955));
#95106=CARTESIAN_POINT('Ctrl Pts',(17.3942426183372,20.8501509875192,-10.4216981395917));
#95107=CARTESIAN_POINT('Ctrl Pts',(17.401039486941,20.8556829683932,-10.4222171682073));
#95108=CARTESIAN_POINT('Ctrl Pts',(17.4133468953465,20.8655735822389,-10.4231574440495));
#95109=CARTESIAN_POINT('Ctrl Pts',(17.4188451985767,20.8699473189401,-10.4235776683576));
#95110=CARTESIAN_POINT('Ctrl Pts',(17.4275606403491,20.8768096355525,-10.4242442034944));
#95111=CARTESIAN_POINT('Ctrl Pts',(17.4307634108325,20.8793164970593,-10.4244892345579));
#95112=CARTESIAN_POINT('Ctrl Pts',(17.4339826888945,20.8818213521995,-10.4247356422545));
#95113=CARTESIAN_POINT('Ctrl Pts',(17.4339920236012,20.8818286152205,-10.424736356746));
#95114=CARTESIAN_POINT('Ctrl Pts',(17.4340107290091,20.8818431690167,-10.4247377884858));
#95115=CARTESIAN_POINT('Ctrl Pts',(17.4340200996542,20.8818504597473,-10.42473850573));
#95116=CARTESIAN_POINT('Ctrl Pts',(17.4340388775657,20.881865069448,-10.4247399430233));
#95117=CARTESIAN_POINT('Ctrl Pts',(17.4340482844276,20.8818723881022,-10.4247406630415));
#95118=CARTESIAN_POINT('Ctrl Pts',(17.4340671346245,20.8818870535317,-10.4247421058715));
#95119=CARTESIAN_POINT('Ctrl Pts',(17.4340765784097,20.8818944006562,-10.4247428287178));
#95120=CARTESIAN_POINT('Ctrl Pts',(17.4340961827591,20.8819096522817,-10.4247443292762));
#95121=CARTESIAN_POINT('Ctrl Pts',(17.4341063432902,20.8819175567368,-10.4247451069859));
#95122=CARTESIAN_POINT('Ctrl Pts',(17.4341268414438,20.8819335031164,-10.4247466759625));
#95123=CARTESIAN_POINT('Ctrl Pts',(17.4341371790578,20.8819415450289,-10.4247474672289));
#95124=CARTESIAN_POINT('Ctrl Pts',(17.4341580351435,20.8819577692376,-10.4247490636072));
#95125=CARTESIAN_POINT('Ctrl Pts',(17.4341685535801,20.8819659515009,-10.4247498687165));
#95126=CARTESIAN_POINT('Ctrl Pts',(17.4341897753024,20.8819824594996,-10.4247514930866));
#95127=CARTESIAN_POINT('Ctrl Pts',(17.434200478368,20.8819907850581,-10.4247523123304));
#95128=CARTESIAN_POINT('Ctrl Pts',(17.4342220730779,20.8820075825311,-10.4247539652551));
#95129=CARTESIAN_POINT('Ctrl Pts',(17.4342329649436,20.882016054612,-10.4247547989528));
#95130=CARTESIAN_POINT('Ctrl Pts',(17.4342549414064,20.8820331483423,-10.4247564811033));
#95131=CARTESIAN_POINT('Ctrl Pts',(17.4342660258785,20.8820417698884,-10.4247573295464));
#95132=CARTESIAN_POINT('Ctrl Pts',(17.4342883914533,20.8820591655634,-10.4247590414862));
#95133=CARTESIAN_POINT('Ctrl Pts',(17.4342996730243,20.8820679400502,-10.4247599050188));
#95134=CARTESIAN_POINT('Ctrl Pts',(17.4343224374474,20.8820856452046,-10.4247616474936));
#95135=CARTESIAN_POINT('Ctrl Pts',(17.4343339199341,20.8820945755815,-10.4247625264078));
#95136=CARTESIAN_POINT('Ctrl Pts',(17.4343570904565,20.8821125958153,-10.4247642999728));
#95137=CARTESIAN_POINT('Ctrl Pts',(17.4343687787576,20.8821216858719,-10.4247651946439));
#95138=CARTESIAN_POINT('Ctrl Pts',(17.4343923656035,20.8821400290955,-10.4247670000821));
#95139=CARTESIAN_POINT('Ctrl Pts',(17.4344042638533,20.8821492820261,-10.4247679108266));
#95140=CARTESIAN_POINT('Ctrl Pts',(17.4344282753377,20.8821679546634,-10.4247697487748));
#95141=CARTESIAN_POINT('Ctrl Pts',(17.4344403884324,20.8821773742537,-10.4247706759677));
#95142=CARTESIAN_POINT('Ctrl Pts',(17.4344648343786,20.8821963838991,-10.4247725471781));
#95143=CARTESIAN_POINT('Ctrl Pts',(17.4344771670345,20.8822059737942,-10.4247734911806));
#95144=CARTESIAN_POINT('Ctrl Pts',(17.4345020565024,20.8822253274464,-10.4247753963471));
#95145=CARTESIAN_POINT('Ctrl Pts',(17.4345146139301,20.8822350916743,-10.4247763575583));
#95146=CARTESIAN_POINT('Ctrl Pts',(17.4345399581839,20.8822547980442,-10.4247782975434));
#95147=CARTESIAN_POINT('Ctrl Pts',(17.434552744946,20.8822647401279,-10.4247792763126));
#95148=CARTESIAN_POINT('Ctrl Pts',(17.4372582990783,20.8843683382574,-10.4249863747096));
#95149=CARTESIAN_POINT('Ctrl Pts',(17.4399560645314,20.8864554386411,-10.4251929608782));
#95150=CARTESIAN_POINT('Ctrl Pts',(17.4462822115505,20.8913252083239,-10.4256775831681));
#95151=CARTESIAN_POINT('Ctrl Pts',(17.4499145604095,20.8941026383864,-10.4259559835004));
#95152=CARTESIAN_POINT('Ctrl Pts',(17.4610851309162,20.9025868670852,-10.4268125018391));
#95153=CARTESIAN_POINT('Ctrl Pts',(17.4686524886779,20.9082548602956,-10.427393229884));
#95154=CARTESIAN_POINT('Ctrl Pts',(17.5750095848097,20.9868103023396,-10.4355590552967));
#95155=CARTESIAN_POINT('Ctrl Pts',(17.6799082885108,21.0510121631218,-10.4436462315541));
#95156=CARTESIAN_POINT('Ctrl Pts',(17.8838341102242,21.1526369452228,-10.4587009219142));
#95157=CARTESIAN_POINT('Ctrl Pts',(17.9812728736565,21.1924492383761,-10.4656428822374));
#95158=CARTESIAN_POINT('Ctrl Pts',(18.1337166699042,21.2418590230281,-10.4759436667052));
#95159=CARTESIAN_POINT('Ctrl Pts',(18.1868090635395,21.2568033505635,-10.4794348464486));
#95160=CARTESIAN_POINT('Ctrl Pts',(18.2737996457122,21.2776596972667,-10.4849952886683));
#95161=CARTESIAN_POINT('Ctrl Pts',(18.3073621497032,21.2848483627479,-10.4871030394444));
#95162=CARTESIAN_POINT('Ctrl Pts',(18.3517084402867,21.2932245365386,-10.4898405320932));
#95163=CARTESIAN_POINT('Ctrl Pts',(18.3623460337021,21.2951495131864,-10.4904936358572));
#95164=CARTESIAN_POINT('Ctrl Pts',(18.3797953896978,21.2981692987134,-10.4915592560542));
#95165=CARTESIAN_POINT('Ctrl Pts',(18.3865984880572,21.2993124236339,-10.4919733025979));
#95166=CARTESIAN_POINT('Ctrl Pts',(18.3997796019268,21.3014610527656,-10.492772831378));
#95167=CARTESIAN_POINT('Ctrl Pts',(18.4061568606474,21.3024706703712,-10.4931584401079));
#95168=CARTESIAN_POINT('Ctrl Pts',(18.4208944206659,21.3047347879344,-10.4940468006514));
#95169=CARTESIAN_POINT('Ctrl Pts',(18.4292578526009,21.3059684228594,-10.4945488866881));
#95170=CARTESIAN_POINT('Ctrl Pts',(18.4517745929107,21.3091520275368,-10.4958952674881));
#95171=CARTESIAN_POINT('Ctrl Pts',(18.4659407761214,21.3110088996141,-10.4967366224294));
#95172=CARTESIAN_POINT('Ctrl Pts',(18.5958916074904,21.3267061572386,-10.5044049443878));
#95173=CARTESIAN_POINT('Ctrl Pts',(18.712622761478,21.3311025274149,-10.510916559998));
#95174=CARTESIAN_POINT('Ctrl Pts',(18.99108064002,21.3185762881616,-10.5261771805903));
#95175=CARTESIAN_POINT('Ctrl Pts',(19.1516331336279,21.2927154600959,-10.5347448739599));
#95176=CARTESIAN_POINT('Ctrl Pts',(19.3396675783229,21.239783538358,-10.5459517653747));
#95177=CARTESIAN_POINT('Ctrl Pts',(19.3714734569208,21.230015397128,-10.5478910473071));
#95178=CARTESIAN_POINT('Ctrl Pts',(19.4099512067565,21.2171984258977,-10.5503055288682));
#95179=CARTESIAN_POINT('Ctrl Pts',(19.416856430259,21.2148585903524,-10.550741548787));
#95180=CARTESIAN_POINT('Ctrl Pts',(19.4276454244655,21.2111404969556,-10.5514272645558));
#95181=CARTESIAN_POINT('Ctrl Pts',(19.4315375671874,21.209786462867,-10.5516755495506));
#95182=CARTESIAN_POINT('Ctrl Pts',(19.4387944069447,21.2072381099467,-10.5521402206967));
#95183=CARTESIAN_POINT('Ctrl Pts',(19.4421600446531,21.2060466406018,-10.5523564373034));
#95184=CARTESIAN_POINT('Ctrl Pts',(19.449821827108,21.203312462588,-10.5528502539361));
#95185=CARTESIAN_POINT('Ctrl Pts',(19.4541159896977,21.2017643751152,-10.553128170088));
#95186=CARTESIAN_POINT('Ctrl Pts',(19.4672516784929,21.1969807697053,-10.5539817547056));
#95187=CARTESIAN_POINT('Ctrl Pts',(19.4760765151719,21.1937001991608,-10.5545600078046));
#95188=CARTESIAN_POINT('Ctrl Pts',(19.5526781134018,21.1646410573214,-10.5596193893968));
#95189=CARTESIAN_POINT('Ctrl Pts',(19.6191040196417,21.1354572821409,-10.5642788191431));
#95190=CARTESIAN_POINT('Ctrl Pts',(19.8068973631509,21.0411704709707,-10.5780020295135));
#95191=CARTESIAN_POINT('Ctrl Pts',(19.9235947535089,20.9675593305937,-10.5872082591452));
#95192=CARTESIAN_POINT('Ctrl Pts',(20.103958599869,20.8275174552415,-10.602012594859));
#95193=CARTESIAN_POINT('Ctrl Pts',(20.1719564835754,20.7673418928319,-10.6077623493589));
#95194=CARTESIAN_POINT('Ctrl Pts',(20.2505685235693,20.6882077023343,-10.6146100491986));
#95195=CARTESIAN_POINT('Ctrl Pts',(20.2650268232026,20.6732173565483,-10.615878929421));
#95196=CARTESIAN_POINT('Ctrl Pts',(20.2853543785955,20.6515096450945,-10.617677168591));
#95197=CARTESIAN_POINT('Ctrl Pts',(20.2914056849412,20.6449651257643,-10.6182143471985));
#95198=CARTESIAN_POINT('Ctrl Pts',(20.3018042242549,20.6335755801998,-10.619140748539));
#95199=CARTESIAN_POINT('Ctrl Pts',(20.30617074213,20.6287484001159,-10.6195307888579));
#95200=CARTESIAN_POINT('Ctrl Pts',(20.3145096746777,20.6194438197673,-10.6202776881177));
#95201=CARTESIAN_POINT('Ctrl Pts',(20.3184854937662,20.6149695674649,-10.6206346884924));
#95202=CARTESIAN_POINT('Ctrl Pts',(20.3288203889694,20.6032392085307,-10.6215650808578));
#95203=CARTESIAN_POINT('Ctrl Pts',(20.3351489772521,20.595956332947,-10.6221371984599));
#95204=CARTESIAN_POINT('Ctrl Pts',(20.3567895491851,20.5707059794782,-10.6241021168707));
#95205=CARTESIAN_POINT('Ctrl Pts',(20.3718510049027,20.5525254090591,-10.6254846366877));
#95206=CARTESIAN_POINT('Ctrl Pts',(20.4897305425364,20.4052886485305,-10.6364378418479));
#95207=CARTESIAN_POINT('Ctrl Pts',(20.5774443167171,20.2648667575945,-10.6453574776964));
#95208=CARTESIAN_POINT('Ctrl Pts',(20.70253723511,20.0002136892172,-10.6612639004333));
#95209=CARTESIAN_POINT('Ctrl Pts',(20.7465429414333,19.8800729594498,-10.6682206367713));
#95210=CARTESIAN_POINT('Ctrl Pts',(20.7825276384248,19.7451963967067,-10.6764580419348));
#95211=CARTESIAN_POINT('Ctrl Pts',(20.7855048900749,19.733646101001,-10.6771668630869));
#95212=CARTESIAN_POINT('Ctrl Pts',(20.7895976349125,19.7171942548811,-10.6781821102731));
#95213=CARTESIAN_POINT('Ctrl Pts',(20.7907935820669,19.7123126967421,-10.67848405377));
#95214=CARTESIAN_POINT('Ctrl Pts',(20.7928242986144,19.7038942219651,-10.6790060496715));
#95215=CARTESIAN_POINT('Ctrl Pts',(20.7936673735354,19.700359292192,-10.6792256252976));
#95216=CARTESIAN_POINT('Ctrl Pts',(20.7952841107707,19.6935022791095,-10.6796523355483));
#95217=CARTESIAN_POINT('Ctrl Pts',(20.796058848062,19.6901804893864,-10.679859401165));
#95218=CARTESIAN_POINT('Ctrl Pts',(20.7981269180614,19.6812154666972,-10.6804191610052));
#95219=CARTESIAN_POINT('Ctrl Pts',(20.7994051233856,19.6755688253309,-10.6807727093471));
#95220=CARTESIAN_POINT('Ctrl Pts',(20.8040603688816,19.6546046675034,-10.6820887777589));
#95221=CARTESIAN_POINT('Ctrl Pts',(20.8072902056153,19.6392554400284,-10.683059191357));
#95222=CARTESIAN_POINT('Ctrl Pts',(20.8366569416978,19.4915690978127,-10.6924524721151));
#95223=CARTESIAN_POINT('Ctrl Pts',(20.8502570013305,19.3570661317236,-10.7014189017867));
#95224=CARTESIAN_POINT('Ctrl Pts',(20.851796465475,19.0660234767047,-10.7206395247686));
#95225=CARTESIAN_POINT('Ctrl Pts',(20.8353383464365,18.9102103424607,-10.7307940198684));
#95226=CARTESIAN_POINT('Ctrl Pts',(20.7973223148153,18.7368243171045,-10.741696039587));
#95227=CARTESIAN_POINT('Ctrl Pts',(20.7924531514088,18.7161139238528,-10.7429926253305));
#95228=CARTESIAN_POINT('Ctrl Pts',(20.7850833571015,18.6867606668681,-10.7448228599915));
#95229=CARTESIAN_POINT('Ctrl Pts',(20.7828386727821,18.6780554315964,-10.7453647141445));
#95230=CARTESIAN_POINT('Ctrl Pts',(20.7788697392067,18.6630590401828,-10.7462966183727));
#95231=CARTESIAN_POINT('Ctrl Pts',(20.7771717528396,18.6567611204135,-10.746687512427));
#95232=CARTESIAN_POINT('Ctrl Pts',(20.7738642628297,18.644715251271,-10.7474342994409));
#95233=CARTESIAN_POINT('Ctrl Pts',(20.7722595064745,18.638966073731,-10.7477903422013));
#95234=CARTESIAN_POINT('Ctrl Pts',(20.7680219782952,18.6240290139886,-10.7487144389166));
#95235=CARTESIAN_POINT('Ctrl Pts',(20.7653512446754,18.6148519714732,-10.7492812526719));
#95236=CARTESIAN_POINT('Ctrl Pts',(20.7560248139155,18.5835954752886,-10.7512088474962));
#95237=CARTESIAN_POINT('Ctrl Pts',(20.7490704023506,18.5616063437684,-10.75255987335));
#95238=CARTESIAN_POINT('Ctrl Pts',(20.6864183968474,18.374213915443,-10.7640406437286));
#95239=CARTESIAN_POINT('Ctrl Pts',(20.61082554301,18.2161727935064,-10.7734290120852));
#95240=CARTESIAN_POINT('Ctrl Pts',(20.4693976187957,17.9953641567839,-10.7876944135508));
#95241=CARTESIAN_POINT('Ctrl Pts',(20.4175745700575,17.9245515434608,-10.7924920188208));
#95242=CARTESIAN_POINT('Ctrl Pts',(20.3372203347245,17.8279537470279,-10.7996647054004));
#95243=CARTESIAN_POINT('Ctrl Pts',(20.3121440866085,17.7994075597901,-10.8018712644293));
#95244=CARTESIAN_POINT('Ctrl Pts',(20.2811604063603,17.765994410635,-10.8045823714871));
#95245=CARTESIAN_POINT('Ctrl Pts',(20.2759757835987,17.7604631493269,-10.8050355405535));
#95246=CARTESIAN_POINT('Ctrl Pts',(20.2678837174925,17.7519224660663,-10.8057423056499));
#95247=CARTESIAN_POINT('Ctrl Pts',(20.2649968124311,17.7488935509174,-10.8059943453365));
#95248=CARTESIAN_POINT('Ctrl Pts',(20.2596346803069,17.7433009431118,-10.8064623364636));
#95249=CARTESIAN_POINT('Ctrl Pts',(20.2571619527434,17.7407349339384,-10.8066780952769));
#95250=CARTESIAN_POINT('Ctrl Pts',(20.2515677533157,17.7349589567297,-10.8071660947011));
#95251=CARTESIAN_POINT('Ctrl Pts',(20.2484425881291,17.7317526597183,-10.8074386214364));
#95252=CARTESIAN_POINT('Ctrl Pts',(20.2392197801862,17.7223502808093,-10.808242552339));
#95253=CARTESIAN_POINT('Ctrl Pts',(20.2330942018934,17.716181903707,-10.8087760776419));
#95254=CARTESIAN_POINT('Ctrl Pts',(20.1895028101289,17.6728233612784,-10.8125686256485));
#95255=CARTESIAN_POINT('Ctrl Pts',(20.1506985209919,17.6370114056801,-10.8159227194899));
#95256=CARTESIAN_POINT('Ctrl Pts',(20.0957757162228,17.5900013321829,-10.820593319889));
#95257=CARTESIAN_POINT('Ctrl Pts',(20.0807765488779,17.5775182348891,-10.821861474106));
#95258=CARTESIAN_POINT('Ctrl Pts',(19.9517444227291,17.4731162590869,-10.8326955011036));
#95259=CARTESIAN_POINT('Ctrl Pts',(19.828615780575,17.3930443130447,-10.8425032285957));
#95260=CARTESIAN_POINT('Ctrl Pts',(19.6432609809496,17.2982159581411,-10.8559541035116));
#95261=CARTESIAN_POINT('Ctrl Pts',(19.5871079499187,17.2725195966533,-10.8598797274755));
#95262=CARTESIAN_POINT('Ctrl Pts',(19.4954182103749,17.2353186860394,-10.8660451208996));
#95263=CARTESIAN_POINT('Ctrl Pts',(19.4605639994366,17.2222367219779,-10.868334641453));
#95264=CARTESIAN_POINT('Ctrl Pts',(19.4148606264061,17.20644476179,-10.8712691199407));
#95265=CARTESIAN_POINT('Ctrl Pts',(19.404311455207,17.2028925685969,-10.8719418488147));
#95266=CARTESIAN_POINT('Ctrl Pts',(19.3871126056886,17.1972518797462,-10.8730312940388));
#95267=CARTESIAN_POINT('Ctrl Pts',(19.3804798687238,17.1951127638984,-10.873449674523));
#95268=CARTESIAN_POINT('Ctrl Pts',(19.3677063568714,17.191062720914,-10.8742520596825));
#95269=CARTESIAN_POINT('Ctrl Pts',(19.3615672099427,17.1891469498021,-10.8746362199113));
#95270=CARTESIAN_POINT('Ctrl Pts',(19.3474936454902,17.1848254549282,-10.8755135452868));
#95271=CARTESIAN_POINT('Ctrl Pts',(19.3395536022625,17.1824382982206,-10.8760060978563));
#95272=CARTESIAN_POINT('Ctrl Pts',(19.3184289104591,17.1762222881013,-10.8773102593886));
#95273=CARTESIAN_POINT('Ctrl Pts',(19.3052205555679,17.172474901218,-10.8781192132815));
#95274=CARTESIAN_POINT('Ctrl Pts',(19.2046461184331,17.1449948741627,-10.8842317136741));
#95275=CARTESIAN_POINT('Ctrl Pts',(19.1158694186432,17.1267582717938,-10.8893516473796));
#95276=CARTESIAN_POINT('Ctrl Pts',(18.8875827937008,17.0949456594772,-10.9021096701358));
#95277=CARTESIAN_POINT('Ctrl Pts',(18.7474098404639,17.0894223146684,-10.909551936079));
#95278=CARTESIAN_POINT('Ctrl Pts',(18.553049335465,17.101036611233,-10.9203112158582));
#95279=CARTESIAN_POINT('Ctrl Pts',(18.4985288706157,17.1064237572823,-10.9233813833286));
#95280=CARTESIAN_POINT('Ctrl Pts',(18.4162441323342,17.1177916078714,-10.9281737958323));
#95281=CARTESIAN_POINT('Ctrl Pts',(18.3882876363909,17.1222269273104,-10.9298302036767));
#95282=CARTESIAN_POINT('Ctrl Pts',(18.3536094120211,17.1284438742993,-10.931929377588));
#95283=CARTESIAN_POINT('Ctrl Pts',(18.3467949373701,17.129700105088,-10.9323440288116));
#95284=CARTESIAN_POINT('Ctrl Pts',(18.3360163096586,17.1317418839388,-10.9330034770276));
#95285=CARTESIAN_POINT('Ctrl Pts',(18.3320479585407,17.1325053796746,-10.9332470357568));
#95286=CARTESIAN_POINT('Ctrl Pts',(18.324564258863,17.1339674485832,-10.933707846386));
#95287=CARTESIAN_POINT('Ctrl Pts',(18.321048489529,17.1346635881807,-10.9339249588606));
#95288=CARTESIAN_POINT('Ctrl Pts',(18.313009880892,17.1362764964414,-10.9344227985276));
#95289=CARTESIAN_POINT('Ctrl Pts',(18.3084882653152,17.1371991273701,-10.9347038569164));
#95290=CARTESIAN_POINT('Ctrl Pts',(18.2964825160983,17.1396898053008,-10.9354527921197));
#95291=CARTESIAN_POINT('Ctrl Pts',(18.2890038796562,17.1412836135805,-10.9359220825106));
#95292=CARTESIAN_POINT('Ctrl Pts',(18.2364179485021,17.152788638724,-10.9392405685189));
#95293=CARTESIAN_POINT('Ctrl Pts',(18.1916403919869,17.1641323302927,-10.9421630057524));
#95294=CARTESIAN_POINT('Ctrl Pts',(18.1424653069691,17.178316859662,-10.94545429852));
#95295=CARTESIAN_POINT('Ctrl Pts',(18.1376620980046,17.1797208099239,-10.945776655514));
#95296=CARTESIAN_POINT('Ctrl Pts',(18.128021654444,17.1825757966011,-10.946425362081));
#95297=CARTESIAN_POINT('Ctrl Pts',(18.1231845415712,17.184027138981,-10.9467517191992));
#95298=CARTESIAN_POINT('Ctrl Pts',(18.0946334810105,17.1927051674271,-10.9486830040868));
#95299=CARTESIAN_POINT('Ctrl Pts',(18.071043300849,17.2003304769855,-10.950298953644));
#95300=CARTESIAN_POINT('Ctrl Pts',(18.010471619697,17.2210915666476,-10.9544924724536));
#95301=CARTESIAN_POINT('Ctrl Pts',(17.9737117390221,17.2348445047715,-10.9570805682199));
#95302=CARTESIAN_POINT('Ctrl Pts',(17.8360961842241,17.2907388688282,-10.9668924698946));
#95303=CARTESIAN_POINT('Ctrl Pts',(17.7381654209825,17.3396499435766,-10.9741188140958));
#95304=CARTESIAN_POINT('Ctrl Pts',(17.5972934727949,17.4242119259793,-10.9846789070399));
#95305=CARTESIAN_POINT('Ctrl Pts',(17.5512600820858,17.4543439569409,-10.9881610777322));
#95306=CARTESIAN_POINT('Ctrl Pts',(17.4785408336145,17.5060997981951,-10.9937088497862));
#95307=CARTESIAN_POINT('Ctrl Pts',(17.4511174762757,17.5266380845204,-10.9958127211388));
#95308=CARTESIAN_POINT('Ctrl Pts',(17.4157162871133,17.5545176561701,-10.9985459883161));
#95309=CARTESIAN_POINT('Ctrl Pts',(17.4072804178645,17.5612664274993,-10.9991986559339));
#95310=CARTESIAN_POINT('Ctrl Pts',(17.3935441175242,17.5724291004065,-11.0002637468903));
#95311=CARTESIAN_POINT('Ctrl Pts',(17.388213020286,17.5768047935323,-11.0006776974077));
#95312=CARTESIAN_POINT('Ctrl Pts',(17.3779321912045,17.5853275872008,-11.0014771667954));
#95313=CARTESIAN_POINT('Ctrl Pts',(17.3729798695991,17.589471430453,-11.0018628114986));
#95314=CARTESIAN_POINT('Ctrl Pts',(17.361585029332,17.5990950153594,-11.0027514350841));
#95315=CARTESIAN_POINT('Ctrl Pts',(17.3551562066668,17.6045908590972,-11.0032537469233));
#95316=CARTESIAN_POINT('Ctrl Pts',(17.3379467271139,17.619482249345,-11.0046011332184));
#95317=CARTESIAN_POINT('Ctrl Pts',(17.3272279297078,17.6289488476746,-11.0054432608958));
#95318=CARTESIAN_POINT('Ctrl Pts',(17.2292160894668,17.7172944772884,-11.0131733304963));
#95319=CARTESIAN_POINT('Ctrl Pts',(17.148539446951,17.8032177076299,-11.0197398030854));
#95320=CARTESIAN_POINT('Ctrl Pts',(16.9737390750565,18.0235917797716,-11.0351343229601));
#95321=CARTESIAN_POINT('Ctrl Pts',(16.887280695856,18.1631105659485,-11.0437794201131));
#95322=CARTESIAN_POINT('Ctrl Pts',(16.8045807992905,18.3392252594405,-11.0549699459295));
#95323=CARTESIAN_POINT('Ctrl Pts',(16.792025146537,18.3675647088137,-11.056779836859));
#95324=CARTESIAN_POINT('Ctrl Pts',(16.7773512486298,18.4027515556841,-11.0590503174971));
#95325=CARTESIAN_POINT('Ctrl Pts',(16.7746389831887,18.4093490245247,-11.0594770223914));
#95326=CARTESIAN_POINT('Ctrl Pts',(16.7704255515091,18.4197471434822,-11.060151292051));
#95327=CARTESIAN_POINT('Ctrl Pts',(16.7689019296574,18.4235387177769,-11.0603975223774));
#95328=CARTESIAN_POINT('Ctrl Pts',(16.7660657190921,18.4306561971514,-11.0608604667148));
#95329=CARTESIAN_POINT('Ctrl Pts',(16.7647505755981,18.4339810244076,-11.0610770241073));
#95330=CARTESIAN_POINT('Ctrl Pts',(16.7617562471194,18.4416074457138,-11.0615744346246));
#95331=CARTESIAN_POINT('Ctrl Pts',(16.7600827142152,18.4459112003731,-11.0618556220099));
#95332=CARTESIAN_POINT('Ctrl Pts',(16.7549425674859,18.4592590260229,-11.0627291387621));
#95333=CARTESIAN_POINT('Ctrl Pts',(16.7515239882663,18.4683212889383,-11.063324227818));
#95334=CARTESIAN_POINT('Ctrl Pts',(16.7472469472449,18.4798992073903,-11.0640868013895));
#95335=CARTESIAN_POINT('Ctrl Pts',(16.7463308326445,18.4823935618772,-11.0642512256825));
#95336=CARTESIAN_POINT('Ctrl Pts',(16.7454194505824,18.4848895411316,-11.0644158872188));
#95337=CARTESIAN_POINT('',(16.617000600774,19.2094051091123,-10.0879364343762));
#95338=CARTESIAN_POINT('Ctrl Pts',(16.7454194500511,18.4848895425866,-10.8441190257052));
#95339=CARTESIAN_POINT('Ctrl Pts',(16.7463456808613,18.4823528974314,-10.8439718529077));
#95340=CARTESIAN_POINT('Ctrl Pts',(16.7472767944397,18.4798179447603,-10.8438247200276));
#95341=CARTESIAN_POINT('Ctrl Pts',(16.8056499912094,18.3218319417938,-10.8346510184629));
#95342=CARTESIAN_POINT('Ctrl Pts',(16.8811330175697,18.1736859260385,-10.8258505658532));
#95343=CARTESIAN_POINT('Ctrl Pts',(16.9808578142822,18.0242493928235,-10.8152891834463));
#95344=CARTESIAN_POINT('Ctrl Pts',(16.9887344673045,18.012695896675,-10.8144605234353));
#95345=CARTESIAN_POINT('Ctrl Pts',(16.9998805543149,17.9966898071256,-10.8132942218365));
#95346=CARTESIAN_POINT('Ctrl Pts',(17.0030540337233,17.992170415238,-10.8129628524692));
#95347=CARTESIAN_POINT('Ctrl Pts',(17.0081863135995,17.984921941929,-10.8124279720849));
#95348=CARTESIAN_POINT('Ctrl Pts',(17.0101340155467,17.9821849805886,-10.8122252190202));
#95349=CARTESIAN_POINT('Ctrl Pts',(17.0142251834924,17.9764648346671,-10.8117997964212));
#95350=CARTESIAN_POINT('Ctrl Pts',(17.0163699017911,17.9734825904479,-10.8115770375478));
#95351=CARTESIAN_POINT('Ctrl Pts',(17.0215923838649,17.9662604264057,-10.8110352698552));
#95352=CARTESIAN_POINT('Ctrl Pts',(17.0246781358047,17.9620263361052,-10.8107157131127));
#95353=CARTESIAN_POINT('Ctrl Pts',(17.0356087281354,17.9471443884301,-10.8095858171662));
#95354=CARTESIAN_POINT('Ctrl Pts',(17.0435374145466,17.9365588887214,-10.8087699406346));
#95355=CARTESIAN_POINT('Ctrl Pts',(17.091565113561,17.8736744015733,-10.8038531925198));
#95356=CARTESIAN_POINT('Ctrl Pts',(17.1339858538914,17.823201322556,-10.799615457748));
#95357=CARTESIAN_POINT('Ctrl Pts',(17.243918256593,17.7041520182491,-10.7890378193802));
#95358=CARTESIAN_POINT('Ctrl Pts',(17.3138862653416,17.6380374290032,-10.7826421490396));
#95359=CARTESIAN_POINT('Ctrl Pts',(17.4967378903779,17.4874345028501,-10.7670586103127));
#95360=CARTESIAN_POINT('Ctrl Pts',(17.6140381139118,17.4090027193463,-10.7580100722682));
#95361=CARTESIAN_POINT('Ctrl Pts',(17.7508859012075,17.3360653790118,-10.7485414236086));
#95362=CARTESIAN_POINT('Ctrl Pts',(17.7635632872765,17.3294724911557,-10.7476734931677));
#95363=CARTESIAN_POINT('Ctrl Pts',(17.7838464468078,17.3191837561465,-10.7462992429362));
#95364=CARTESIAN_POINT('Ctrl Pts',(17.7914091199717,17.3154043386634,-10.7457899954639));
#95365=CARTESIAN_POINT('Ctrl Pts',(17.8047871228633,17.308818589694,-10.7448946326345));
#95366=CARTESIAN_POINT('Ctrl Pts',(17.8105929932058,17.3059933884664,-10.7445078612206));
#95367=CARTESIAN_POINT('Ctrl Pts',(17.8226282411554,17.3002048509659,-10.7437097896492));
#95368=CARTESIAN_POINT('Ctrl Pts',(17.8288593662753,17.2972453084829,-10.7432986249091));
#95369=CARTESIAN_POINT('Ctrl Pts',(17.8448911680343,17.2897266408971,-10.7422458868943));
#95370=CARTESIAN_POINT('Ctrl Pts',(17.8547125740576,17.285211988661,-10.7416058550837));
#95371=CARTESIAN_POINT('Ctrl Pts',(17.8958499553497,17.2666824897977,-10.7389449658021));
#95372=CARTESIAN_POINT('Ctrl Pts',(17.9274707415219,17.2533542634829,-10.7369476421261));
#95373=CARTESIAN_POINT('Ctrl Pts',(18.0106938051536,17.2206345696118,-10.7318029468363));
#95374=CARTESIAN_POINT('Ctrl Pts',(18.0627549203165,17.2024788807158,-10.7286949766252));
#95375=CARTESIAN_POINT('Ctrl Pts',(18.2200494142554,17.1544247381263,-10.7195498487507));
#95376=CARTESIAN_POINT('Ctrl Pts',(18.3269517784088,17.1306251201954,-10.7136614180894));
#95377=CARTESIAN_POINT('Ctrl Pts',(18.4810888913437,17.1086507754174,-10.7051846655704));
#95378=CARTESIAN_POINT('Ctrl Pts',(18.5271649999029,17.1036188467924,-10.7026508028881));
#95379=CARTESIAN_POINT('Ctrl Pts',(18.5947027911534,17.0984794406683,-10.6988935419683));
#95380=CARTESIAN_POINT('Ctrl Pts',(18.6160608743801,17.0971794906358,-10.6976990306905));
#95381=CARTESIAN_POINT('Ctrl Pts',(18.6892330596353,17.0938383129726,-10.6935744655786));
#95382=CARTESIAN_POINT('Ctrl Pts',(18.7410966161713,17.0933771860091,-10.6905959233844));
#95383=CARTESIAN_POINT('Ctrl Pts',(18.8015718362507,17.0950609745616,-10.6870052852223));
#95384=CARTESIAN_POINT('Ctrl Pts',(18.8102219541795,17.0953549162636,-10.6864888831743));
#95385=CARTESIAN_POINT('Ctrl Pts',(18.8233354689785,17.0958810558833,-10.685701429351));
#95386=CARTESIAN_POINT('Ctrl Pts',(18.8278004538525,17.096074363531,-10.6854325036307));
#95387=CARTESIAN_POINT('Ctrl Pts',(18.8358239937517,17.0964471938743,-10.6849477412303));
#95388=CARTESIAN_POINT('Ctrl Pts',(18.8393827338521,17.0966215630365,-10.6847321958953));
#95389=CARTESIAN_POINT('Ctrl Pts',(18.8471262686733,17.0970205748798,-10.6842620107358));
#95390=CARTESIAN_POINT('Ctrl Pts',(18.8513107879042,17.0972486568108,-10.6840071857044));
#95391=CARTESIAN_POINT('Ctrl Pts',(18.8630928837328,17.0979259471869,-10.6832876526075));
#95392=CARTESIAN_POINT('Ctrl Pts',(18.8706886647821,17.0984036991928,-10.6828213908528));
#95393=CARTESIAN_POINT('Ctrl Pts',(18.9167087457112,17.1015474518372,-10.6799826831708));
#95394=CARTESIAN_POINT('Ctrl Pts',(18.9550544199134,17.1052205597344,-10.6775591249822));
#95395=CARTESIAN_POINT('Ctrl Pts',(19.0823756916008,17.120932276181,-10.6693637707954));
#95396=CARTESIAN_POINT('Ctrl Pts',(19.1706807197682,17.1375833322489,-10.6634408411964));
#95397=CARTESIAN_POINT('Ctrl Pts',(19.4238615944747,17.20221812311,-10.6461739133023));
#95398=CARTESIAN_POINT('Ctrl Pts',(19.5843273030891,17.2647011797319,-10.6349279670057));
#95399=CARTESIAN_POINT('Ctrl Pts',(19.7560012174503,17.3568847258749,-10.6229309459337));
#95400=CARTESIAN_POINT('Ctrl Pts',(19.7763099310615,17.3682249150958,-10.6215108773086));
#95401=CARTESIAN_POINT('Ctrl Pts',(19.8047233172305,17.3847107159517,-10.6195221822124));
#95402=CARTESIAN_POINT('Ctrl Pts',(19.8129856408882,17.3895799598714,-10.6189436533945));
#95403=CARTESIAN_POINT('Ctrl Pts',(19.8263413871064,17.3975736871088,-10.6180080132134));
#95404=CARTESIAN_POINT('Ctrl Pts',(19.8314551022912,17.4006638439605,-10.6176496577185));
#95405=CARTESIAN_POINT('Ctrl Pts',(19.8421196563331,17.407170100265,-10.6169020475993));
#95406=CARTESIAN_POINT('Ctrl Pts',(19.8476679465778,17.410590272699,-10.6165129473782));
#95407=CARTESIAN_POINT('Ctrl Pts',(19.8608074120459,17.4187739065306,-10.6155910686919));
#95408=CARTESIAN_POINT('Ctrl Pts',(19.8683843481337,17.4235600797718,-10.6150591348975));
#95409=CARTESIAN_POINT('Ctrl Pts',(19.893705234678,17.4397805477699,-10.6132801934133));
#95410=CARTESIAN_POINT('Ctrl Pts',(19.9113088721777,17.4514323126798,-10.612041282077));
#95411=CARTESIAN_POINT('Ctrl Pts',(20.0055364870751,17.5158484304989,-10.6053929023444));
#95412=CARTESIAN_POINT('Ctrl Pts',(20.0787976271102,17.5733595863709,-10.6001690193662));
#95413=CARTESIAN_POINT('Ctrl Pts',(20.2631903066744,17.7388569404021,-10.5865243612946));
#95414=CARTESIAN_POINT('Ctrl Pts',(20.3666500472961,17.8545061476902,-10.5783423827433));
#95415=CARTESIAN_POINT('Ctrl Pts',(20.4877612361527,18.0240340843417,-10.5666284270531));
#95416=CARTESIAN_POINT('Ctrl Pts',(20.5172708705414,18.0688482910641,-10.5635510417338));
#95417=CARTESIAN_POINT('Ctrl Pts',(20.5495711994075,18.1222086343617,-10.5598496860012));
#95418=CARTESIAN_POINT('Ctrl Pts',(20.5540515795039,18.1297148109813,-10.5593281862634));
#95419=CARTESIAN_POINT('Ctrl Pts',(20.5607615168274,18.1411161270856,-10.5585344774732));
#95420=CARTESIAN_POINT('Ctrl Pts',(20.5630254499802,18.1449910678816,-10.5582644454499));
#95421=CARTESIAN_POINT('Ctrl Pts',(20.5670652689543,18.151956363566,-10.5577785085781));
#95422=CARTESIAN_POINT('Ctrl Pts',(20.5688456856062,18.1550440284572,-10.5575629013832));
#95423=CARTESIAN_POINT('Ctrl Pts',(20.5726953637035,18.1617594168982,-10.5570935408109));
#95424=CARTESIAN_POINT('Ctrl Pts',(20.5747616630726,18.1653887238561,-10.5568396074713));
#95425=CARTESIAN_POINT('Ctrl Pts',(20.5805304866881,18.1755913467433,-10.5561250539674));
#95426=CARTESIAN_POINT('Ctrl Pts',(20.5842085882237,18.1821782984234,-10.5556629136313));
#95427=CARTESIAN_POINT('Ctrl Pts',(20.605885280426,18.221490332854,-10.5529005931958));
#95428=CARTESIAN_POINT('Ctrl Pts',(20.6230493304123,18.2546652699205,-10.5505523783761));
#95429=CARTESIAN_POINT('Ctrl Pts',(20.676436359367,18.3649035356381,-10.5427354543226));
#95430=CARTESIAN_POINT('Ctrl Pts',(20.7088879644602,18.4436969970264,-10.5371293825934));
#95431=CARTESIAN_POINT('Ctrl Pts',(20.7942920234098,18.6927187536137,-10.5197380965397));
#95432=CARTESIAN_POINT('Ctrl Pts',(20.8305935381181,18.8678692505629,-10.508032042151));
#95433=CARTESIAN_POINT('Ctrl Pts',(20.8463035046377,19.068234531975,-10.4956638611662));
#95434=CARTESIAN_POINT('Ctrl Pts',(20.8477176651531,19.0909759597103,-10.4942732103255));
#95435=CARTESIAN_POINT('Ctrl Pts',(20.8492014991643,19.1232384179958,-10.4923182623713));
#95436=CARTESIAN_POINT('Ctrl Pts',(20.849574477277,19.1327432874682,-10.4917445112734));
#95437=CARTESIAN_POINT('Ctrl Pts',(20.8500769567745,19.1482079464258,-10.4908144957193));
#95438=CARTESIAN_POINT('Ctrl Pts',(20.8502453676407,19.1541662595599,-10.4904570164647));
#95439=CARTESIAN_POINT('Ctrl Pts',(20.8505455380383,19.166653342831,-10.4897095677839));
#95440=CARTESIAN_POINT('Ctrl Pts',(20.8506722596,19.1731821800572,-10.4893197600837));
#95441=CARTESIAN_POINT('Ctrl Pts',(20.8509022271688,19.1887402617858,-10.4883931749867));
#95442=CARTESIAN_POINT('Ctrl Pts',(20.8509779171904,19.1977698332267,-10.4878572657998));
#95443=CARTESIAN_POINT('Ctrl Pts',(20.8510385098232,19.2283093128937,-10.4860508192928));
#95444=CARTESIAN_POINT('Ctrl Pts',(20.8507533655752,19.2498188599572,-10.4847887297042));
#95445=CARTESIAN_POINT('Ctrl Pts',(20.8450120733732,19.4512312258627,-10.4730571815745));
#95446=CARTESIAN_POINT('Ctrl Pts',(20.8169638006571,19.6297502361542,-10.4633898141733));
#95447=CARTESIAN_POINT('Ctrl Pts',(20.7331540340856,19.9177188354101,-10.4470657321036));
#95448=CARTESIAN_POINT('Ctrl Pts',(20.689927413938,20.0297844315691,-10.4404845547594));
#95449=CARTESIAN_POINT('Ctrl Pts',(20.6332938716225,20.146126906848,-10.4328161010472));
#95450=CARTESIAN_POINT('Ctrl Pts',(20.629071614573,20.1546541266213,-10.4322489339741));
#95451=CARTESIAN_POINT('Ctrl Pts',(20.6227301663004,20.1672470268566,-10.4314033205938));
#95452=CARTESIAN_POINT('Ctrl Pts',(20.6206549544595,20.1713348891776,-10.4311275586822));
#95453=CARTESIAN_POINT('Ctrl Pts',(20.6169391562285,20.1785959356094,-10.4306354320642));
#95454=CARTESIAN_POINT('Ctrl Pts',(20.6153038003953,20.1817717399348,-10.4304193975591));
#95455=CARTESIAN_POINT('Ctrl Pts',(20.6117705938852,20.1885906455286,-10.4299538232286));
#95456=CARTESIAN_POINT('Ctrl Pts',(20.6098702035568,20.1922323130788,-10.4297041286948));
#95457=CARTESIAN_POINT('Ctrl Pts',(20.6045953937572,20.2022689623246,-10.4290130952983));
#95458=CARTESIAN_POINT('Ctrl Pts',(20.6011988278623,20.2086521520893,-10.4285703901153));
#95459=CARTESIAN_POINT('Ctrl Pts',(20.5824139318691,20.2435227717658,-10.4261348021302));
#95460=CARTESIAN_POINT('Ctrl Pts',(20.5664071964543,20.2716700423081,-10.4241059367913));
#95461=CARTESIAN_POINT('Ctrl Pts',(20.4660409327737,20.4391039225393,-10.4117033358881));
#95462=CARTESIAN_POINT('Ctrl Pts',(20.366487666859,20.5686409554826,-10.4007371245855));
#95463=CARTESIAN_POINT('Ctrl Pts',(20.1716614589363,20.769358343412,-10.3824655434921));
#95464=CARTESIAN_POINT('Ctrl Pts',(20.083434795197,20.8463546256413,-10.3750199444763));
#95465=CARTESIAN_POINT('Ctrl Pts',(19.9777952958741,20.9241450474022,-10.3670096145457));
#95466=CARTESIAN_POINT('Ctrl Pts',(19.966217442339,20.9324914701889,-10.3661427030888));
#95467=CARTESIAN_POINT('Ctrl Pts',(19.9476520770016,20.9455918914904,-10.3647697562727));
#95468=CARTESIAN_POINT('Ctrl Pts',(19.9407191318255,20.950422126499,-10.364260801866));
#95469=CARTESIAN_POINT('Ctrl Pts',(19.9284383166171,20.9588694992475,-10.3633657798626));
#95470=CARTESIAN_POINT('Ctrl Pts',(19.9231025057767,20.962503899736,-10.3629790577809));
#95471=CARTESIAN_POINT('Ctrl Pts',(19.9120295316824,20.9699721526607,-10.3621809208398));
#95472=CARTESIAN_POINT('Ctrl Pts',(19.9062900761022,20.9738024820034,-10.3617696422219));
#95473=CARTESIAN_POINT('Ctrl Pts',(19.8915045302492,20.9835657365504,-10.360716266342));
#95474=CARTESIAN_POINT('Ctrl Pts',(19.8824314348382,20.989457554734,-10.3600757142129));
#95475=CARTESIAN_POINT('Ctrl Pts',(19.8443316550008,21.0137853508032,-10.3574097625365));
#95476=CARTESIAN_POINT('Ctrl Pts',(19.8149021775307,21.0315828972413,-10.355408011231));
#95477=CARTESIAN_POINT('Ctrl Pts',(19.7370616172996,21.0761039464869,-10.3502493270476));
#95478=CARTESIAN_POINT('Ctrl Pts',(19.6880134213877,21.1016624187991,-10.3471320771683));
#95479=CARTESIAN_POINT('Ctrl Pts',(19.4673801613852,21.2058567861411,-10.3335668218609));
#95480=CARTESIAN_POINT('Ctrl Pts',(19.2867569893165,21.2632538229222,-10.3237191112559));
#95481=CARTESIAN_POINT('Ctrl Pts',(19.0604411030488,21.3030841887266,-10.3106515664));
#95482=CARTESIAN_POINT('Ctrl Pts',(19.0197450698734,21.3090298619439,-10.3082707374228));
#95483=CARTESIAN_POINT('Ctrl Pts',(18.9715637294868,21.3146413900157,-10.3053885547431));
#95484=CARTESIAN_POINT('Ctrl Pts',(18.964218284229,21.3154579257725,-10.3049474213742));
#95485=CARTESIAN_POINT('Ctrl Pts',(18.9523064932537,21.3167189563785,-10.3042290304884));
#95486=CARTESIAN_POINT('Ctrl Pts',(18.9477426418276,21.3171871071688,-10.3039530695453));
#95487=CARTESIAN_POINT('Ctrl Pts',(18.939622305831,21.3179934101271,-10.3034607249753));
#95488=CARTESIAN_POINT('Ctrl Pts',(18.9360664511866,21.3183373987221,-10.3032446726777));
#95489=CARTESIAN_POINT('Ctrl Pts',(18.9284222596688,21.3190573617101,-10.3027792164663));
#95490=CARTESIAN_POINT('Ctrl Pts',(18.9243337551308,21.3194304390496,-10.3025296586692));
#95491=CARTESIAN_POINT('Ctrl Pts',(18.9130516005739,21.3204268562338,-10.3018393801654));
#95492=CARTESIAN_POINT('Ctrl Pts',(18.9058558854201,21.3210252815201,-10.3013972979557));
#95493=CARTESIAN_POINT('Ctrl Pts',(18.8665230637097,21.3240938303984,-10.2989713643165));
#95494=CARTESIAN_POINT('Ctrl Pts',(18.8343376672896,21.3258664234142,-10.2969518591124));
#95495=CARTESIAN_POINT('Ctrl Pts',(18.639249404319,21.3321477476314,-10.2845523662688));
#95496=CARTESIAN_POINT('Ctrl Pts',(18.4763162096868,21.3185683610775,-10.273577526453));
#95497=CARTESIAN_POINT('Ctrl Pts',(18.2019753830702,21.2633884481375,-10.2552983262862));
#95498=CARTESIAN_POINT('Ctrl Pts',(18.0894871427162,21.2308909697044,-10.2478532317566));
#95499=CARTESIAN_POINT('Ctrl Pts',(17.9668770779023,21.1841740787605,-10.2398415196094));
#95500=CARTESIAN_POINT('Ctrl Pts',(17.9535648266366,21.1789467672255,-10.2389728172653));
#95501=CARTESIAN_POINT('Ctrl Pts',(17.9324653004991,21.1704138567701,-10.2375975797614));
#95502=CARTESIAN_POINT('Ctrl Pts',(17.9246432817456,21.1671958599451,-10.2370881103717));
#95503=CARTESIAN_POINT('Ctrl Pts',(17.910883833508,21.161438533487,-10.2361924893891));
#95504=CARTESIAN_POINT('Ctrl Pts',(17.9049383828698,21.158918769581,-10.2358056805486));
#95505=CARTESIAN_POINT('Ctrl Pts',(17.8935292333466,21.1540217168015,-10.2350637328261));
#95506=CARTESIAN_POINT('Ctrl Pts',(17.8880638675277,21.1516484901846,-10.2347084601706));
#95507=CARTESIAN_POINT('Ctrl Pts',(17.8736594669946,21.1453212519478,-10.2337724528282));
#95508=CARTESIAN_POINT('Ctrl Pts',(17.8647376036873,21.1413283217344,-10.2331930536703));
#95509=CARTESIAN_POINT('Ctrl Pts',(17.831697139405,21.1262657191009,-10.2310483636955));
#95510=CARTESIAN_POINT('Ctrl Pts',(17.8077590499509,21.1148043550685,-10.2294965619977));
#95511=CARTESIAN_POINT('Ctrl Pts',(17.7489357811437,21.0852680325913,-10.2256835572129));
#95512=CARTESIAN_POINT('Ctrl Pts',(17.7143256919695,21.0666661180826,-10.2234404200608));
#95513=CARTESIAN_POINT('Ctrl Pts',(17.5863680018275,20.9932309106059,-10.2151165739654));
#95514=CARTESIAN_POINT('Ctrl Pts',(17.4967505080721,20.9322269100176,-10.2092331319849));
#95515=CARTESIAN_POINT('Ctrl Pts',(17.305801095767,20.7795940084054,-10.1959580068644));
#95516=CARTESIAN_POINT('Ctrl Pts',(17.2078821672328,20.6844969836559,-10.1886008864898));
#95517=CARTESIAN_POINT('Ctrl Pts',(17.1096885924245,20.5687721019393,-10.1797012671102));
#95518=CARTESIAN_POINT('Ctrl Pts',(17.0997222558615,20.5567595820042,-10.1787778696874));
#95519=CARTESIAN_POINT('Ctrl Pts',(17.0862501011173,20.5401511031376,-10.1775000006378));
#95520=CARTESIAN_POINT('Ctrl Pts',(17.082628647919,20.535649025208,-10.1771534901056));
#95521=CARTESIAN_POINT('Ctrl Pts',(17.0769001140311,20.5284674899228,-10.1766004625432));
#95522=CARTESIAN_POINT('Ctrl Pts',(17.0747809658554,20.5257976328828,-10.1763948024152));
#95523=CARTESIAN_POINT('Ctrl Pts',(17.0704149445373,20.5202696363774,-10.1759688219611));
#95524=CARTESIAN_POINT('Ctrl Pts',(17.0681689892963,20.517410831438,-10.1757484367202));
#95525=CARTESIAN_POINT('Ctrl Pts',(17.0628305404511,20.510579540437,-10.1752216244526));
#95526=CARTESIAN_POINT('Ctrl Pts',(17.059744841147,20.5066017931078,-10.1749147206601));
#95527=CARTESIAN_POINT('Ctrl Pts',(17.0493660175254,20.493123549008,-10.1738744091635));
#95528=CARTESIAN_POINT('Ctrl Pts',(17.0421394942459,20.4835723805295,-10.1731365473979));
#95529=CARTESIAN_POINT('Ctrl Pts',(16.9597944676103,20.3727972400555,-10.1645761840224));
#95530=CARTESIAN_POINT('Ctrl Pts',(16.8937877008371,20.2651300396035,-10.1562460925395));
#95531=CARTESIAN_POINT('Ctrl Pts',(16.8040456883625,20.0843347708155,-10.1429073629733));
#95532=CARTESIAN_POINT('Ctrl Pts',(16.7740074419759,20.0146587587977,-10.1379034860672));
#95533=CARTESIAN_POINT('Ctrl Pts',(16.7335752731302,19.9050267144563,-10.1303131071387));
#95534=CARTESIAN_POINT('Ctrl Pts',(16.7205007735365,19.8661284806985,-10.1276720524118));
#95535=CARTESIAN_POINT('Ctrl Pts',(16.7056936940796,19.8174321089819,-10.1244341631383));
#95536=CARTESIAN_POINT('Ctrl Pts',(16.7028889868685,19.807971046537,-10.123808231091));
#95537=CARTESIAN_POINT('Ctrl Pts',(16.6846210540898,19.7447287996249,-10.1196453076624));
#95538=CARTESIAN_POINT('Ctrl Pts',(16.6712283474928,19.6903688847012,-10.1161694891358));
#95539=CARTESIAN_POINT('Ctrl Pts',(16.6575926826235,19.6237545460312,-10.1120304221958));
#95540=CARTESIAN_POINT('Ctrl Pts',(16.6552811246771,19.6119507571611,-10.111301489832));
#95541=CARTESIAN_POINT('Ctrl Pts',(16.6516247786829,19.5923977958541,-10.1101012848126));
#95542=CARTESIAN_POINT('Ctrl Pts',(16.6502223738101,19.5846598028042,-10.1096281849467));
#95543=CARTESIAN_POINT('Ctrl Pts',(16.647762545748,19.5706426376986,-10.1087745130955));
#95544=CARTESIAN_POINT('Ctrl Pts',(16.646690278268,19.5643661971801,-10.1083934731164));
#95545=CARTESIAN_POINT('Ctrl Pts',(16.6446635349805,19.5521716130033,-10.1076554515411));
#95546=CARTESIAN_POINT('Ctrl Pts',(16.6437058478971,19.5462540714129,-10.1072983713889));
#95547=CARTESIAN_POINT('Ctrl Pts',(16.6416603185898,19.5332651754798,-10.106516856433));
#95548=CARTESIAN_POINT('Ctrl Pts',(16.6405831595346,19.5261921948508,-10.1060927626622));
#95549=CARTESIAN_POINT('Ctrl Pts',(16.6380227879121,19.508787616514,-10.1050527316809));
#95550=CARTESIAN_POINT('Ctrl Pts',(16.6365800762816,19.4984501827135,-10.10443807039));
#95551=CARTESIAN_POINT('Ctrl Pts',(16.6230153915459,19.3957106312585,-10.098358525497));
#95552=CARTESIAN_POINT('Ctrl Pts',(16.6169303822837,19.3026105459037,-10.0930911649182));
#95553=CARTESIAN_POINT('Ctrl Pts',(16.617000600774,19.2094051091123,-10.0879364343762));
#95554=CARTESIAN_POINT('Ctrl Pts',(16.6170005988921,19.2094076090818,-10.0879365726371));
#95555=CARTESIAN_POINT('Ctrl Pts',(16.6171166072579,19.0551806300102,-10.079407039861));
#95556=CARTESIAN_POINT('Ctrl Pts',(16.6340851386937,18.901431767422,-10.0712484902641));
#95557=CARTESIAN_POINT('Ctrl Pts',(16.6803058095911,18.6938498832741,-10.0593799989335));
#95558=CARTESIAN_POINT('Ctrl Pts',(16.6953621981461,18.6373635760974,-10.0560550010929));
#95559=CARTESIAN_POINT('Ctrl Pts',(16.716425838712,18.5697218254495,-10.0518778646937));
#95560=CARTESIAN_POINT('Ctrl Pts',(16.7202219175506,18.5578989270259,-10.0511403713423));
#95561=CARTESIAN_POINT('Ctrl Pts',(16.7257260431972,18.5412606411189,-10.0500911539455));
#95562=CARTESIAN_POINT('Ctrl Pts',(16.7273479344961,18.536416735182,-10.0497843303886));
#95563=CARTESIAN_POINT('Ctrl Pts',(16.7301583328951,18.5281230810269,-10.0492565739232));
#95564=CARTESIAN_POINT('Ctrl Pts',(16.7313382697674,18.5246704090759,-10.0490361462883));
#95565=CARTESIAN_POINT('Ctrl Pts',(16.7336315060848,18.5180163227447,-10.0486099114122));
#95566=CARTESIAN_POINT('Ctrl Pts',(16.7347435721344,18.5148145192164,-10.0484041827799));
#95567=CARTESIAN_POINT('Ctrl Pts',(16.7377395838904,18.5062549352212,-10.0478525254537));
#95568=CARTESIAN_POINT('Ctrl Pts',(16.7396373932051,18.500902086918,-10.0475057854285));
#95569=CARTESIAN_POINT('Ctrl Pts',(16.7428347657553,18.4919976967176,-10.0469261397184));
#95570=CARTESIAN_POINT('Ctrl Pts',(16.7441223562984,18.4884418608032,-10.0466939075207));
#95571=CARTESIAN_POINT('Ctrl Pts',(16.7454194503153,18.4848895418633,-10.0464611586511));
#95572=CARTESIAN_POINT('Origin',(18.734,19.211,0.));
#95573=CARTESIAN_POINT('',(16.7454193052938,18.48488993903,-9.24346979856369));
#95574=CARTESIAN_POINT('',(16.7454194503191,18.4848895418526,-9.46634969422496));
#95575=CARTESIAN_POINT('',(16.7454194503191,18.4848895418526,0.));
#95576=CARTESIAN_POINT('',(16.6163914501725,19.212893456819,-9.51094371951111));
#95577=CARTESIAN_POINT('Ctrl Pts',(16.7454194503191,18.4848895418526,-9.46634969422496));
#95578=CARTESIAN_POINT('Ctrl Pts',(16.7207383638393,18.552483016052,-9.47066127900277));
#95579=CARTESIAN_POINT('Ctrl Pts',(16.6995057450598,18.6213417166538,-9.47497286378058));
#95580=CARTESIAN_POINT('Ctrl Pts',(16.6818386275887,18.6910743307134,-9.47928444855839));
#95581=CARTESIAN_POINT('Ctrl Pts',(16.6641689584331,18.7608170163443,-9.48359665606395));
#95582=CARTESIAN_POINT('Ctrl Pts',(16.6500659226405,18.8314333804341,-9.48790886356951));
#95583=CARTESIAN_POINT('Ctrl Pts',(16.6395956397896,18.9025208662947,-9.49222107107507));
#95584=CARTESIAN_POINT('Ctrl Pts',(16.6291143285382,18.9736832289539,-9.49653782065002));
#95585=CARTESIAN_POINT('Ctrl Pts',(16.6222734603225,19.0453172089163,-9.50085457022496));
#95586=CARTESIAN_POINT('Ctrl Pts',(16.6190872658805,19.1170152828417,-9.5051713197999));
#95587=CARTESIAN_POINT('Ctrl Pts',(16.6176670680779,19.14897361084,-9.50709544539002));
#95588=CARTESIAN_POINT('Ctrl Pts',(16.6169722855427,19.1809446693594,-9.50901957098014));
#95589=CARTESIAN_POINT('Ctrl Pts',(16.6170008459316,19.2128925310153,-9.51094369657026));
#95590=CARTESIAN_POINT('Ctrl Pts',(16.616352496962,19.2128935159973,-9.51094372097751));
#95591=CARTESIAN_POINT('Ctrl Pts',(16.6150297892913,19.3558822368191,-9.51955279572481));
#95592=CARTESIAN_POINT('Ctrl Pts',(16.6934794697575,20.2015184257048,-9.57055380603261));
#95593=CARTESIAN_POINT('Ctrl Pts',(17.8308508198777,21.5456632002202,-9.66394675190086));
#95594=CARTESIAN_POINT('Ctrl Pts',(20.2082247613025,21.2341144439155,-9.79112255858231));
#95595=CARTESIAN_POINT('Ctrl Pts',(21.2330889849398,19.0664837539622,-9.91829836526374));
#95596=CARTESIAN_POINT('Ctrl Pts',(19.9651941758507,17.0314377500589,-10.0454741719452));
#95597=CARTESIAN_POINT('Ctrl Pts',(17.7787242164569,16.9991228464334,-10.1614588018767));
#95598=CARTESIAN_POINT('Ctrl Pts',(16.9288259028377,17.999326025981,-10.2350514962479));
#95599=CARTESIAN_POINT('Ctrl Pts',(16.746026985005,18.4851209024697,-10.2662522550585));
#95600=CARTESIAN_POINT('Ctrl Pts',(16.7454194503153,18.4848895418633,-10.0464611586511));
#95601=CARTESIAN_POINT('Ctrl Pts',(16.7492540692639,18.4743877668629,-10.0457730795959));
#95602=CARTESIAN_POINT('Ctrl Pts',(16.7531717467079,18.4639167294962,-10.0450804854191));
#95603=CARTESIAN_POINT('Ctrl Pts',(16.8130754566754,18.3075922481247,-10.0346477479531));
#95604=CARTESIAN_POINT('Ctrl Pts',(16.8849512981194,18.168354599542,-10.0241793135717));
#95605=CARTESIAN_POINT('Ctrl Pts',(17.008579340344,17.9825467946946,-10.0094871214254));
#95606=CARTESIAN_POINT('Ctrl Pts',(17.0483025349942,17.9285808762599,-10.0051142817485));
#95607=CARTESIAN_POINT('Ctrl Pts',(17.1238637070005,17.8355188273289,-9.99742294536467));
#95608=CARTESIAN_POINT('Ctrl Pts',(17.1587373763441,17.7957135494896,-9.99407827262933));
#95609=CARTESIAN_POINT('Ctrl Pts',(17.2102742753661,17.7411567222447,-9.98941730963709));
#95610=CARTESIAN_POINT('Ctrl Pts',(17.2257324572609,17.7252986765136,-9.98805258656972));
#95611=CARTESIAN_POINT('Ctrl Pts',(17.2533937989356,17.6977985785221,-9.98566773739921));
#95612=CARTESIAN_POINT('Ctrl Pts',(17.2654923617964,17.6860545560752,-9.98464318061443));
#95613=CARTESIAN_POINT('Ctrl Pts',(17.2836655776281,17.6688307694723,-9.98313106070535));
#95614=CARTESIAN_POINT('Ctrl Pts',(17.2896335483837,17.663239867202,-9.9826386954157));
#95615=CARTESIAN_POINT('Ctrl Pts',(17.3003433859421,17.6533225906868,-9.98176252567437));
#95616=CARTESIAN_POINT('Ctrl Pts',(17.3050727895254,17.6489829619723,-9.98137815627133));
#95617=CARTESIAN_POINT('Ctrl Pts',(17.3143686781063,17.6405307471637,-9.98062757758779));
#95618=CARTESIAN_POINT('Ctrl Pts',(17.3189334744815,17.6364164062244,-9.98026129592865));
#95619=CARTESIAN_POINT('Ctrl Pts',(17.3313367527173,17.6253345876643,-9.97927218697373));
#95620=CARTESIAN_POINT('Ctrl Pts',(17.3392092648349,17.6184053258125,-9.97865096555531));
#95621=CARTESIAN_POINT('Ctrl Pts',(17.3689940318019,17.5925795012267,-9.97632483663104));
#95622=CARTESIAN_POINT('Ctrl Pts',(17.391242049636,17.5740737920539,-9.97463603941793));
#95623=CARTESIAN_POINT('Ctrl Pts',(17.4163835301155,17.5540189405063,-9.97277793205473));
#95624=CARTESIAN_POINT('Ctrl Pts',(17.4189083850078,17.5520143347317,-9.97259188201449));
#95625=CARTESIAN_POINT('Ctrl Pts',(17.5510070719603,17.4476257986891,-9.9628864276219));
#95626=CARTESIAN_POINT('Ctrl Pts',(17.6921098443273,17.3607484032004,-9.9540113924558));
#95627=CARTESIAN_POINT('Ctrl Pts',(17.9201176582946,17.254798050159,-9.94032893772111));
#95628=CARTESIAN_POINT('Ctrl Pts',(18.0004913157635,17.2232643051149,-9.93560410729653));
#95629=CARTESIAN_POINT('Ctrl Pts',(18.1183659381789,17.1851421289355,-9.92852953561705));
#95630=CARTESIAN_POINT('Ctrl Pts',(18.1544750131813,17.1745187681236,-9.92634309891679));
#95631=CARTESIAN_POINT('Ctrl Pts',(18.1981532580054,17.1629242111301,-9.92365429506091));
#95632=CARTESIAN_POINT('Ctrl Pts',(18.2054713226853,17.1610235120352,-9.92320232876492));
#95633=CARTESIAN_POINT('Ctrl Pts',(18.2168505578096,17.1581329983979,-9.92249703890991));
#95634=CARTESIAN_POINT('Ctrl Pts',(18.2209048278413,17.1571159196686,-9.92224526128661));
#95635=CARTESIAN_POINT('Ctrl Pts',(18.2284214636035,17.1552538956571,-9.92177750816716));
#95636=CARTESIAN_POINT('Ctrl Pts',(18.2318829607817,17.1544056840669,-9.92156172370697));
#95637=CARTESIAN_POINT('Ctrl Pts',(18.2397035969862,17.1525102223619,-9.92107334683157));
#95638=CARTESIAN_POINT('Ctrl Pts',(18.2440639056234,17.1514680820039,-9.92080046631611));
#95639=CARTESIAN_POINT('Ctrl Pts',(18.2569148476295,17.1484397478758,-9.91999454489041));
#95640=CARTESIAN_POINT('Ctrl Pts',(18.2654143600164,17.1464921825656,-9.91945936741901));
#95641=CARTESIAN_POINT('Ctrl Pts',(18.3259979202234,17.1330035481429,-9.9156306099981));
#95642=CARTESIAN_POINT('Ctrl Pts',(18.3784854394883,17.1233833416842,-9.91223995785051));
#95643=CARTESIAN_POINT('Ctrl Pts',(18.4487909540028,17.1132254620416,-9.90764899083443));
#95644=CARTESIAN_POINT('Ctrl Pts',(18.466337582523,17.1109145213346,-9.90649910286534));
#95645=CARTESIAN_POINT('Ctrl Pts',(18.6323989769895,17.0911587229751,-9.89558919544303));
#95646=CARTESIAN_POINT('Ctrl Pts',(18.7823572736117,17.089274972707,-9.88557070750275));
#95647=CARTESIAN_POINT('Ctrl Pts',(18.9915058265951,17.1088484888464,-9.87201180486261));
#95648=CARTESIAN_POINT('Ctrl Pts',(19.0514851450734,17.1170672228508,-9.86816628965925));
#95649=CARTESIAN_POINT('Ctrl Pts',(19.1471454487915,17.134380980075,-9.8621115742965));
#95650=CARTESIAN_POINT('Ctrl Pts',(19.1830819600255,17.1418549172568,-9.8598548080031));
#95651=CARTESIAN_POINT('Ctrl Pts',(19.2295884228364,17.1527959847386,-9.85695568532932));
#95652=CARTESIAN_POINT('Ctrl Pts',(19.2403490877864,17.1554168073544,-9.85628637957847));
#95653=CARTESIAN_POINT('Ctrl Pts',(19.257834825701,17.1598211996922,-9.85520109132212));
#95654=CARTESIAN_POINT('Ctrl Pts',(19.2645724428938,17.1615536649894,-9.85478346835702));
#95655=CARTESIAN_POINT('Ctrl Pts',(19.2775258510273,17.1649525763561,-9.85398160591887));
#95656=CARTESIAN_POINT('Ctrl Pts',(19.2837428139334,17.1666142119269,-9.8535972158727));
#95657=CARTESIAN_POINT('Ctrl Pts',(19.2979781359502,17.1704885812375,-9.85271807302966));
#95658=CARTESIAN_POINT('Ctrl Pts',(19.3059912566813,17.1727202858234,-9.85222394158878));
#95659=CARTESIAN_POINT('Ctrl Pts',(19.3272832161136,17.1787856797925,-9.85091281873817));
#95660=CARTESIAN_POINT('Ctrl Pts',(19.3405381561843,17.1827023156396,-9.85009852836811));
#95661=CARTESIAN_POINT('Ctrl Pts',(19.4430477054654,17.214087105365,-9.84381412368992));
#95662=CARTESIAN_POINT('Ctrl Pts',(19.5304405352526,17.2473056883049,-9.83854010890437));
#95663=CARTESIAN_POINT('Ctrl Pts',(19.7430328055279,17.3446509004538,-9.82561620829409));
#95664=CARTESIAN_POINT('Ctrl Pts',(19.8645634469252,17.4156643549884,-9.81815228126884));
#95665=CARTESIAN_POINT('Ctrl Pts',(20.0204612238266,17.5289062587479,-9.80748377970363));
#95666=CARTESIAN_POINT('Ctrl Pts',(20.061601687841,17.5611833884103,-9.80454707106764));
#95667=CARTESIAN_POINT('Ctrl Pts',(20.1224477667727,17.6126712996269,-9.79994373655688));
#95668=CARTESIAN_POINT('Ctrl Pts',(20.1430453062894,17.6307996967275,-9.79833692891243));
#95669=CARTESIAN_POINT('Ctrl Pts',(20.1683434615907,17.6539531536821,-9.79629325551477));
#95670=CARTESIAN_POINT('Ctrl Pts',(20.1733807068907,17.658608546427,-9.79588275767558));
#95671=CARTESIAN_POINT('Ctrl Pts',(20.1813381984575,17.6660348403788,-9.79522841857553));
#95672=CARTESIAN_POINT('Ctrl Pts',(20.1842733679834,17.6687897800061,-9.79498578314173));
#95673=CARTESIAN_POINT('Ctrl Pts',(20.1898094649726,17.6740157214674,-9.7945256771551));
#95674=CARTESIAN_POINT('Ctrl Pts',(20.1924119755468,17.6764849692458,-9.79430833996899));
#95675=CARTESIAN_POINT('Ctrl Pts',(20.1983673842118,17.6821642630852,-9.79380861865852));
#95676=CARTESIAN_POINT('Ctrl Pts',(20.2017160071915,17.6853787273052,-9.79352589431809));
#95677=CARTESIAN_POINT('Ctrl Pts',(20.2106189760876,17.6939814490588,-9.79276962965887));
#95678=CARTESIAN_POINT('Ctrl Pts',(20.2161543345916,17.6993891345004,-9.79229463244431));
#95679=CARTESIAN_POINT('Ctrl Pts',(20.2556991517151,17.7384478838658,-9.78886744999699));
#95680=CARTESIAN_POINT('Ctrl Pts',(20.2885861840402,17.7732103543356,-9.78583671952136));
#95681=CARTESIAN_POINT('Ctrl Pts',(20.3224481120616,17.8115242172951,-9.78254440456992));
#95682=CARTESIAN_POINT('Ctrl Pts',(20.3246257969968,17.8139998407904,-9.782331879831));
#95683=CARTESIAN_POINT('Ctrl Pts',(20.4269986198787,17.9309284304711,-9.77230397843741));
#95684=CARTESIAN_POINT('Ctrl Pts',(20.5145729492168,18.0558419406547,-9.76208554370552));
#95685=CARTESIAN_POINT('Ctrl Pts',(20.6351908030188,18.2746685108814,-9.74582900641361));
#95686=CARTESIAN_POINT('Ctrl Pts',(20.6763948395662,18.3634447106208,-9.73961186505247));
#95687=CARTESIAN_POINT('Ctrl Pts',(20.7190611821095,18.4750035762942,-9.73227315357857));
#95688=CARTESIAN_POINT('Ctrl Pts',(20.7264914836894,18.4953629588576,-9.73095197618365));
#95689=CARTESIAN_POINT('Ctrl Pts',(20.7365820843569,18.5243880131049,-9.72909340797457));
#95690=CARTESIAN_POINT('Ctrl Pts',(20.7395011965821,18.5329616680246,-9.7285474622993));
#95691=CARTESIAN_POINT('Ctrl Pts',(20.744431741942,18.5477535024243,-9.72761072930052));
#95692=CARTESIAN_POINT('Ctrl Pts',(20.7464695496129,18.5539626959433,-9.72721907476441));
#95693=CARTESIAN_POINT('Ctrl Pts',(20.7503093568817,18.5658480478928,-9.72647232728343));
#95694=CARTESIAN_POINT('Ctrl Pts',(20.752116217565,18.5715225590581,-9.72611707735638));
#95695=CARTESIAN_POINT('Ctrl Pts',(20.7567377754345,18.5862514157768,-9.72519824456619));
#95696=CARTESIAN_POINT('Ctrl Pts',(20.7595156508851,18.5953172455518,-9.72463587349696));
#95697=CARTESIAN_POINT('Ctrl Pts',(20.7687082540731,18.6260537846362,-9.72273973530326));
#95698=CARTESIAN_POINT('Ctrl Pts',(20.7748369877245,18.6478089120701,-9.72141528972613));
#95699=CARTESIAN_POINT('Ctrl Pts',(20.8267306204514,18.844000015531,-9.70961825731916));
#95700=CARTESIAN_POINT('Ctrl Pts',(20.8503804708857,19.0235151551127,-9.69994615606126));
#95701=CARTESIAN_POINT('Ctrl Pts',(20.8512697721163,19.2875215914897,-9.68556915647499));
#95702=CARTESIAN_POINT('Ctrl Pts',(20.8465929758142,19.3711110805741,-9.68097955105233));
#95703=CARTESIAN_POINT('Ctrl Pts',(20.8327384784995,19.4909142006391,-9.67408773917421));
#95704=CARTESIAN_POINT('Ctrl Pts',(20.8275318223549,19.5275111297979,-9.67193934244312));
#95705=CARTESIAN_POINT('Ctrl Pts',(20.8201163022152,19.5713669674984,-9.66929271173391));
#95706=CARTESIAN_POINT('Ctrl Pts',(20.8188227543208,19.57877663989,-9.66884305623137));
#95707=CARTESIAN_POINT('Ctrl Pts',(20.8167505002429,19.5902845297706,-9.6681406010822));
#95708=CARTESIAN_POINT('Ctrl Pts',(20.8159991064496,19.594387689994,-9.66788932746214));
#95709=CARTESIAN_POINT('Ctrl Pts',(20.8145831201494,19.6019930786009,-9.6674220294971));
#95710=CARTESIAN_POINT('Ctrl Pts',(20.8139218071814,19.6054958590183,-9.66720619311979));
#95711=CARTESIAN_POINT('Ctrl Pts',(20.8124067153879,19.6134111384847,-9.66671707865762));
#95712=CARTESIAN_POINT('Ctrl Pts',(20.8115477348622,19.6178225749063,-9.66644350862493));
#95713=CARTESIAN_POINT('Ctrl Pts',(20.8089707809303,19.6308359239727,-9.66563370134964));
#95714=CARTESIAN_POINT('Ctrl Pts',(20.8072134085111,19.6394298092203,-9.6650952972764));
#95715=CARTESIAN_POINT('Ctrl Pts',(20.7941141569381,19.7015191875241,-9.66118046218243));
#95716=CARTESIAN_POINT('Ctrl Pts',(20.7807576067344,19.754563801033,-9.65770205393585));
#95717=CARTESIAN_POINT('Ctrl Pts',(20.7569589868554,19.8356737064115,-9.65223431796181));
#95718=CARTESIAN_POINT('Ctrl Pts',(20.7479487979251,19.864138911725,-9.65028631284497));
#95719=CARTESIAN_POINT('Ctrl Pts',(20.6966418051746,20.0150578664716,-9.63983132792635));
#95720=CARTESIAN_POINT('Ctrl Pts',(20.6437692710081,20.1336358389845,-9.63118811452694));
#95721=CARTESIAN_POINT('Ctrl Pts',(20.5373135348998,20.3234306219613,-9.61709969325426));
#95722=CARTESIAN_POINT('Ctrl Pts',(20.4894871086742,20.3974695509572,-9.61152497183786));
#95723=CARTESIAN_POINT('Ctrl Pts',(20.4250081502671,20.4848134022355,-9.60486236547195));
#95724=CARTESIAN_POINT('Ctrl Pts',(20.412595144485,20.5011269454122,-9.60361372204411));
#95725=CARTESIAN_POINT('Ctrl Pts',(20.3944820200499,20.5242276649228,-9.60183890369111));
#95726=CARTESIAN_POINT('Ctrl Pts',(20.3889734814306,20.5311629514248,-9.60130518516355));
#95727=CARTESIAN_POINT('Ctrl Pts',(20.3793475301045,20.5431271495623,-9.60038284499195));
#95728=CARTESIAN_POINT('Ctrl Pts',(20.3752502133798,20.5481720068729,-9.59999342518898));
#95729=CARTESIAN_POINT('Ctrl Pts',(20.3673267166262,20.5578365960045,-9.59924639392123));
#95730=CARTESIAN_POINT('Ctrl Pts',(20.3635040118203,20.5624590841693,-9.59888864733137));
#95731=CARTESIAN_POINT('Ctrl Pts',(20.3534366916731,20.5745278662587,-9.59795339129189));
#95732=CARTESIAN_POINT('Ctrl Pts',(20.3471603133288,20.5819475732814,-9.59737718280924));
#95733=CARTESIAN_POINT('Ctrl Pts',(20.3251921072876,20.6075578367705,-9.59538375582243));
#95734=CARTESIAN_POINT('Ctrl Pts',(20.309241548751,20.6255247421433,-9.59397722769793));
#95735=CARTESIAN_POINT('Ctrl Pts',(20.1932797773993,20.7517507599045,-9.58402729141683));
#95736=CARTESIAN_POINT('Ctrl Pts',(20.0825083053685,20.8495793783059,-9.57598757869103));
#95737=CARTESIAN_POINT('Ctrl Pts',(19.9242566551874,20.9623362202565,-9.56543471879967));
#95738=CARTESIAN_POINT('Ctrl Pts',(19.8851594843455,20.9882791564423,-9.56289016444519));
#95739=CARTESIAN_POINT('Ctrl Pts',(19.7844807513065,21.0503677683157,-9.55641965473239));
#95740=CARTESIAN_POINT('Ctrl Pts',(19.7218766022878,21.0847347369993,-9.55247023570512));
#95741=CARTESIAN_POINT('Ctrl Pts',(19.6274569851025,21.1305182915925,-9.5464520746851));
#95742=CARTESIAN_POINT('Ctrl Pts',(19.5969097691629,21.1444431205361,-9.54449580956827));
#95743=CARTESIAN_POINT('Ctrl Pts',(19.5593240133737,21.1605083277931,-9.54206245036514));
#95744=CARTESIAN_POINT('Ctrl Pts',(19.5525868589147,21.1633467924668,-9.54162526040247));
#95745=CARTESIAN_POINT('Ctrl Pts',(19.542025319404,21.1677322508391,-9.54093810751089));
#95746=CARTESIAN_POINT('Ctrl Pts',(19.5382108106522,21.1693030893185,-9.5406895651657));
#95747=CARTESIAN_POINT('Ctrl Pts',(19.5310869305714,21.1722124231457,-9.54022467301018));
#95748=CARTESIAN_POINT('Ctrl Pts',(19.5277787567277,21.1735537007471,-9.54000849434791));
#95749=CARTESIAN_POINT('Ctrl Pts',(19.5202385334113,21.1765886515958,-9.53951510622221));
#95750=CARTESIAN_POINT('Ctrl Pts',(19.5160044132099,21.178277020535,-9.53923758281343));
#95751=CARTESIAN_POINT('Ctrl Pts',(19.5049816719668,21.1826311657002,-9.5385139515651));
#95752=CARTESIAN_POINT('Ctrl Pts',(19.4981847353083,21.1852755326612,-9.53806660820199));
#95753=CARTESIAN_POINT('Ctrl Pts',(19.4548183114908,21.2018898647136,-9.53520585950243));
#95754=CARTESIAN_POINT('Ctrl Pts',(19.4178833833633,21.2148773819395,-9.53273980900384));
#95755=CARTESIAN_POINT('Ctrl Pts',(19.3688627141953,21.2306015937719,-9.52944739524212));
#95756=CARTESIAN_POINT('Ctrl Pts',(19.3570803642369,21.2342676818479,-9.52865458386929));
#95757=CARTESIAN_POINT('Ctrl Pts',(19.3221509550216,21.2448019569476,-9.52630119425002));
#95758=CARTESIAN_POINT('Ctrl Pts',(19.2989180848994,21.251377279152,-9.52473193265296));
#95759=CARTESIAN_POINT('Ctrl Pts',(19.1362200052563,21.2944319928249,-9.51373620565939));
#95760=CARTESIAN_POINT('Ctrl Pts',(18.9934449913382,21.3169827021489,-9.50408906971004));
#95761=CARTESIAN_POINT('Ctrl Pts',(18.7877688404288,21.3282194917069,-9.49078080512738));
#95762=CARTESIAN_POINT('Ctrl Pts',(18.7259288403398,21.3288870251516,-9.48684921389634));
#95763=CARTESIAN_POINT('Ctrl Pts',(18.6269048136485,21.3256176602687,-9.48067559158439));
#95764=CARTESIAN_POINT('Ctrl Pts',(18.5897034140495,21.3234052641623,-9.47838364469238));
#95765=CARTESIAN_POINT('Ctrl Pts',(18.5414838613437,21.3192576985587,-9.47544654961667));
#95766=CARTESIAN_POINT('Ctrl Pts',(18.5303974115057,21.3182159311648,-9.47477356915816));
#95767=CARTESIAN_POINT('Ctrl Pts',(18.5123855102357,21.3163799177615,-9.47368381845691));
#95768=CARTESIAN_POINT('Ctrl Pts',(18.5054549613428,21.3156388638672,-9.4732653823345));
#95769=CARTESIAN_POINT('Ctrl Pts',(18.4921372994051,21.314148303961,-9.47246295852408));
#95770=CARTESIAN_POINT('Ctrl Pts',(18.4857497040293,21.3134038970551,-9.47207881491793));
#95771=CARTESIAN_POINT('Ctrl Pts',(18.4711367174029,21.3116333812185,-9.47120162169463));
#95772=CARTESIAN_POINT('Ctrl Pts',(18.4629137289167,21.3105880415549,-9.47070918401676));
#95773=CARTESIAN_POINT('Ctrl Pts',(18.4410945242486,21.3076839741336,-9.46940552840154));
#95774=CARTESIAN_POINT('Ctrl Pts',(18.4275097400249,21.3057412820877,-9.46859696220938));
#95775=CARTESIAN_POINT('Ctrl Pts',(18.3247121551399,21.290019271718,-9.4625001283872));
#95776=CARTESIAN_POINT('Ctrl Pts',(18.2364381087653,21.2706778149047,-9.45739434951155));
#95777=CARTESIAN_POINT('Ctrl Pts',(18.0155894319129,21.2072546253011,-9.44467437854784));
#95778=CARTESIAN_POINT('Ctrl Pts',(17.8856587089938,21.1555980236109,-9.4372549163098));
#95779=CARTESIAN_POINT('Ctrl Pts',(17.7126396959872,21.0661467104089,-9.42649617802183));
#95780=CARTESIAN_POINT('Ctrl Pts',(17.6645407027813,21.0388408435081,-9.42339806931545));
#95781=CARTESIAN_POINT('Ctrl Pts',(17.5933680501374,20.9946645116841,-9.418566180751));
#95782=CARTESIAN_POINT('Ctrl Pts',(17.5694739381421,20.9791570084667,-9.41689953416408));
#95783=CARTESIAN_POINT('Ctrl Pts',(17.5401543141232,20.9592762057995,-9.41478891286748));
#95784=CARTESIAN_POINT('Ctrl Pts',(17.5344266243157,20.9553511477776,-9.41437342075452));
#95785=CARTESIAN_POINT('Ctrl Pts',(17.5253935827218,20.9490954762626,-9.41371293829239));
#95786=CARTESIAN_POINT('Ctrl Pts',(17.5220753641855,20.9467834061213,-9.41346919281735));
#95787=CARTESIAN_POINT('Ctrl Pts',(17.5158296068885,20.9424048441377,-9.41300823757602));
#95788=CARTESIAN_POINT('Ctrl Pts',(17.5129006824989,20.9403404225424,-9.41279116845311));
#95789=CARTESIAN_POINT('Ctrl Pts',(17.5062161342057,20.9356034402861,-9.41229369997646));
#95790=CARTESIAN_POINT('Ctrl Pts',(17.5024639928413,20.9329260464654,-9.4120129712115));
#95791=CARTESIAN_POINT('Ctrl Pts',(17.492525460807,20.9257851652729,-9.41126548329841));
#95792=CARTESIAN_POINT('Ctrl Pts',(17.4863544668134,20.9213005040056,-9.41079731905449));
#95793=CARTESIAN_POINT('Ctrl Pts',(17.443297529304,20.88965260017,-9.40750318760877));
#95794=CARTESIAN_POINT('Ctrl Pts',(17.4072803239944,20.8613337943083,-9.40460515677022));
#95795=CARTESIAN_POINT('Ctrl Pts',(17.3434297895935,20.8076893097437,-9.39924370791611));
#95796=CARTESIAN_POINT('Ctrl Pts',(17.3152969431568,20.7827454222939,-9.39679632998763));
#95797=CARTESIAN_POINT('Ctrl Pts',(17.192180401704,20.6675850159885,-9.38574620590467));
#95798=CARTESIAN_POINT('Ctrl Pts',(17.1050205714435,20.5694098384852,-9.37700301638097));
#95799=CARTESIAN_POINT('Ctrl Pts',(16.9752026493684,20.3925789203905,-9.36279856210357));
#95800=CARTESIAN_POINT('Ctrl Pts',(16.9274171308401,20.318139840831,-9.35720316584235));
#95801=CARTESIAN_POINT('Ctrl Pts',(16.8744284018121,20.2229803454949,-9.350518661249));
#95802=CARTESIAN_POINT('Ctrl Pts',(16.8646987126618,20.2048930990092,-9.34926760830961));
#95803=CARTESIAN_POINT('Ctrl Pts',(16.8511486070113,20.1788006979053,-9.3474899990882));
#95804=CARTESIAN_POINT('Ctrl Pts',(16.8471131270901,20.1709091058635,-9.34695586658156));
#95805=CARTESIAN_POINT('Ctrl Pts',(16.8402042019883,20.1571864130415,-9.34603304104757));
#95806=CARTESIAN_POINT('Ctrl Pts',(16.8373078557513,20.1513670369589,-9.34564354754152));
#95807=CARTESIAN_POINT('Ctrl Pts',(16.8317911215019,20.140153562817,-9.34489653437175));
#95808=CARTESIAN_POINT('Ctrl Pts',(16.8291667639353,20.1347614977118,-9.34453887882267));
#95809=CARTESIAN_POINT('Ctrl Pts',(16.8223533123523,20.1206099257183,-9.34360421428273));
#95810=CARTESIAN_POINT('Ctrl Pts',(16.8182014765784,20.1118325581299,-9.3430285030187));
#95811=CARTESIAN_POINT('Ctrl Pts',(16.8040088680341,20.0812861163131,-9.34103852825398));
#95812=CARTESIAN_POINT('Ctrl Pts',(16.7942773423047,20.0593747838186,-9.33963490520103));
#95813=CARTESIAN_POINT('Ctrl Pts',(16.7250855532629,19.896165311332,-9.32934404558491));
#95814=CARTESIAN_POINT('Ctrl Pts',(16.6807559351145,19.7489446285711,-9.32100721195334));
#95815=CARTESIAN_POINT('Ctrl Pts',(16.6289120186581,19.4702808470904,-9.30561469617625));
#95816=CARTESIAN_POINT('Ctrl Pts',(16.6169601914145,19.3404434587236,-9.29857228888663));
#95817=CARTESIAN_POINT('Ctrl Pts',(16.6170011042399,19.207075682044,-9.29078130925382));
#95818=CARTESIAN_POINT('Ctrl Pts',(16.6170097080016,19.2038008171236,-9.29058964995036));
#95819=CARTESIAN_POINT('Ctrl Pts',(16.6171033847899,19.1848671289577,-9.28947947365972));
#95820=CARTESIAN_POINT('Ctrl Pts',(16.6173545929795,19.169210108466,-9.288553141191));
#95821=CARTESIAN_POINT('Ctrl Pts',(16.6179364383876,19.1477744042352,-9.28727182822806));
#95822=CARTESIAN_POINT('Ctrl Pts',(16.6181171280736,19.1419917161239,-9.28692486431782));
#95823=CARTESIAN_POINT('Ctrl Pts',(16.6184419928259,19.1328018696173,-9.28637129196932));
#95824=CARTESIAN_POINT('Ctrl Pts',(16.6185707023715,19.129394144399,-9.28616554346365));
#95825=CARTESIAN_POINT('Ctrl Pts',(16.6188536013079,19.1223550755574,-9.28573953431244));
#95826=CARTESIAN_POINT('Ctrl Pts',(16.6190089085143,19.1187238238374,-9.28551920944345));
#95827=CARTESIAN_POINT('Ctrl Pts',(16.6194013861738,19.1100693729792,-9.28499279542433));
#95828=CARTESIAN_POINT('Ctrl Pts',(16.6196471049501,19.1050465995675,-9.28468623140508));
#95829=CARTESIAN_POINT('Ctrl Pts',(16.6205368678634,19.0880965206623,-9.28364825192569));
#95830=CARTESIAN_POINT('Ctrl Pts',(16.6212639477807,19.0761740577846,-9.28291240896649));
#95831=CARTESIAN_POINT('Ctrl Pts',(16.6311137078558,18.9344158113935,-9.27409997408766));
#95832=CARTESIAN_POINT('Ctrl Pts',(16.6520897229059,18.8056948566674,-9.26548333018932));
#95833=CARTESIAN_POINT('Ctrl Pts',(16.7018392867629,18.6137972733215,-9.25238337418594));
#95834=CARTESIAN_POINT('Ctrl Pts',(16.7220915832289,18.5487770275629,-9.24789461432881));
#95835=CARTESIAN_POINT('Ctrl Pts',(16.7454193052938,18.48488993903,-9.24346979856369));
#95836=CARTESIAN_POINT('Origin',(18.734,19.211,0.));
#95837=CARTESIAN_POINT('',(16.7454194503191,18.4848895418526,-8.44448864899009));
#95838=CARTESIAN_POINT('',(16.745419494333,18.4848894213129,-8.66553665550751));
#95839=CARTESIAN_POINT('',(16.7454194503191,18.4848895418526,0.));
#95840=CARTESIAN_POINT('',(16.6170000013281,19.2110749873286,-8.71094372102528));
#95841=CARTESIAN_POINT('Ctrl Pts',(16.745419494333,18.4848894213129,-8.66553665550751));
#95842=CARTESIAN_POINT('Ctrl Pts',(16.733311422067,18.5180494897324,-8.6678589517768));
#95843=CARTESIAN_POINT('Ctrl Pts',(16.7220302073804,18.5515194592593,-8.67019227608761));
#95844=CARTESIAN_POINT('Ctrl Pts',(16.6746521894853,18.7046488048368,-8.68078506136069));
#95845=CARTESIAN_POINT('Ctrl Pts',(16.6483548014453,18.827078406676,-8.68900850976821));
#95846=CARTESIAN_POINT('Ctrl Pts',(16.6297591080332,18.9774166931212,-8.69860359135708));
#95847=CARTESIAN_POINT('Ctrl Pts',(16.6270006266104,19.0037691441327,-8.70026803505595));
#95848=CARTESIAN_POINT('Ctrl Pts',(16.6216845094513,19.0657772309175,-8.70414332149744));
#95849=CARTESIAN_POINT('Ctrl Pts',(16.61953371278,19.1014602866226,-8.70634145746368));
#95850=CARTESIAN_POINT('Ctrl Pts',(16.6178981538474,19.1483376779776,-8.70918908236397));
#95851=CARTESIAN_POINT('Ctrl Pts',(16.6175971722505,19.1594959412993,-8.70986394166662));
#95852=CARTESIAN_POINT('Ctrl Pts',(16.6172522425656,19.177592504778,-8.71095375470374));
#95853=CARTESIAN_POINT('Ctrl Pts',(16.6171541291415,19.1845294474272,-8.71137039777877));
#95854=CARTESIAN_POINT('Ctrl Pts',(16.6170502016127,19.195792596711,-8.71204510585635));
#95855=CARTESIAN_POINT('Ctrl Pts',(16.6170235457636,19.2001185182293,-8.71230382138551));
#95856=CARTESIAN_POINT('Ctrl Pts',(16.6170034293859,19.2066147842418,-8.71269170733863));
#95857=CARTESIAN_POINT('Ctrl Pts',(16.6170000462397,19.2087850663916,-8.71282118744952));
#95858=CARTESIAN_POINT('Ctrl Pts',(16.6170000004708,19.2109553548739,-8.71295056330574));
#95859=CARTESIAN_POINT('Ctrl Pts',(16.6170000013281,19.2110749873285,-8.71094372102528));
#95860=CARTESIAN_POINT('Ctrl Pts',(16.6170027209272,19.2878531769883,-8.71553605185446));
#95861=CARTESIAN_POINT('Ctrl Pts',(16.6211865549027,19.36454594767,-8.72012838268363));
#95862=CARTESIAN_POINT('Ctrl Pts',(16.6294980530144,19.4406966589526,-8.72472071351281));
#95863=CARTESIAN_POINT('Ctrl Pts',(16.6378338109209,19.5170696407095,-8.72932644854445));
#95864=CARTESIAN_POINT('Ctrl Pts',(16.650321266275,19.5928969954323,-8.73393218357609));
#95865=CARTESIAN_POINT('Ctrl Pts',(16.6668554550742,19.6677301505086,-8.73853791860773));
#95866=CARTESIAN_POINT('Ctrl Pts',(16.6834151174018,19.7426785978757,-8.74315074950138));
#95867=CARTESIAN_POINT('Ctrl Pts',(16.7040338351224,19.8166294002008,-8.74776358039503));
#95868=CARTESIAN_POINT('Ctrl Pts',(16.7285569647206,19.8891498597281,-8.75237641128868));
#95869=CARTESIAN_POINT('Ctrl Pts',(16.7531478646363,19.9618707314645,-8.75700198986258));
#95870=CARTESIAN_POINT('Ctrl Pts',(16.781664593162,20.0331529809713,-8.76162756843648));
#95871=CARTESIAN_POINT('Ctrl Pts',(16.8139044122089,20.1025839465498,-8.76625314701037));
#95872=CARTESIAN_POINT('Ctrl Pts',(16.8312431022427,20.1399241682537,-8.76874079971719));
#95873=CARTESIAN_POINT('Ctrl Pts',(16.8496578472074,20.1767293760275,-8.77122845242401));
#95874=CARTESIAN_POINT('Ctrl Pts',(16.8691118619909,20.2129387370059,-8.77371610513083));
#95875=CARTESIAN_POINT('Ctrl Pts',(16.9034286623952,20.2768118977539,-8.77810431406173));
#95876=CARTESIAN_POINT('Ctrl Pts',(16.9410977666969,20.3390446523179,-8.78249252299263));
#95877=CARTESIAN_POINT('Ctrl Pts',(16.9819381659417,20.3992627359453,-8.78688073192353));
#95878=CARTESIAN_POINT('Ctrl Pts',(17.0227179512625,20.4593914459522,-8.79126242802479));
#95879=CARTESIAN_POINT('Ctrl Pts',(17.0666594195114,20.5175110248671,-8.79564412412605));
#95880=CARTESIAN_POINT('Ctrl Pts',(17.1135357879718,20.5732719029386,-8.80002582022732));
#95881=CARTESIAN_POINT('Ctrl Pts',(17.1603570729688,20.6289672575408,-8.80440236748696));
#95882=CARTESIAN_POINT('Ctrl Pts',(17.2101060983649,20.6823090498175,-8.8087789147466));
#95883=CARTESIAN_POINT('Ctrl Pts',(17.2625139124398,20.7329782173594,-8.81315546200624));
#95884=CARTESIAN_POINT('Ctrl Pts',(17.3148884902406,20.7836152512518,-8.81752923372322));
#95885=CARTESIAN_POINT('Ctrl Pts',(17.3699181652065,20.831582688923,-8.82190300544019));
#95886=CARTESIAN_POINT('Ctrl Pts',(17.4272959551551,20.8765970518664,-8.82627677715716));
#95887=CARTESIAN_POINT('Ctrl Pts',(17.4846562848495,20.9215977167879,-8.83064921792071));
#95888=CARTESIAN_POINT('Ctrl Pts',(17.5443629316526,20.9636467934747,-8.83502165868427));
#95889=CARTESIAN_POINT('Ctrl Pts',(17.6060758346833,21.0025010681813,-8.83939409944782));
#95890=CARTESIAN_POINT('Ctrl Pts',(17.6677903157196,21.0413563363958,-8.84376665201516));
#95891=CARTESIAN_POINT('Ctrl Pts',(17.7315107455601,21.0770163851239,-8.8481392045825));
#95892=CARTESIAN_POINT('Ctrl Pts',(17.7968695201135,21.1092822402551,-8.85251175714984));
#95893=CARTESIAN_POINT('Ctrl Pts',(17.8622961264685,21.1415815821077,-8.85688884771717));
#95894=CARTESIAN_POINT('Ctrl Pts',(17.9293640389054,21.1704794832203,-8.8612659382845));
#95895=CARTESIAN_POINT('Ctrl Pts',(17.9976833250388,21.1958241116467,-8.86564302885182));
#95896=CARTESIAN_POINT('Ctrl Pts',(18.06603992287,21.2211825817153,-8.87002250991077));
#95897=CARTESIAN_POINT('Ctrl Pts',(18.1356487944357,21.2429837711611,-8.87440199096971));
#95898=CARTESIAN_POINT('Ctrl Pts',(18.2061050046721,21.2611258190433,-8.87878147202865));
#95899=CARTESIAN_POINT('Ctrl Pts',(18.2766860980683,21.2793000235835,-8.88316871568837));
#95900=CARTESIAN_POINT('Ctrl Pts',(18.3481170562227,21.2938020386139,-8.88755595934809));
#95901=CARTESIAN_POINT('Ctrl Pts',(18.4199835016908,21.3045812950038,-8.89194320300781));
#95902=CARTESIAN_POINT('Ctrl Pts',(18.4688457595749,21.3119101506622,-8.89492610594263));
#95903=CARTESIAN_POINT('Ctrl Pts',(18.517909182163,21.3175191746183,-8.89790900887744));
#95904=CARTESIAN_POINT('Ctrl Pts',(18.5670433388758,21.3214062341896,-8.90089191181226));
#95905=CARTESIAN_POINT('Ctrl Pts',(18.6393255921071,21.3271245662635,-8.90528012074316));
#95906=CARTESIAN_POINT('Ctrl Pts',(18.712043061856,21.3291362205188,-8.90966832967406));
#95907=CARTESIAN_POINT('Ctrl Pts',(18.78478307398,21.3273908144285,-8.91405653860495));
#95908=CARTESIAN_POINT('Ctrl Pts',(18.8574151278656,21.3256479988102,-8.91843823470622));
#95909=CARTESIAN_POINT('Ctrl Pts',(18.9300691794575,21.3201592036426,-8.92281993080748));
#95910=CARTESIAN_POINT('Ctrl Pts',(19.0023285427324,21.3109259018249,-8.92720162690875));
#95911=CARTESIAN_POINT('Ctrl Pts',(19.0745029955047,21.3017034498717,-8.93157817416839));
#95912=CARTESIAN_POINT('Ctrl Pts',(19.1462832051698,21.2887452929198,-8.93595472142802));
#95913=CARTESIAN_POINT('Ctrl Pts',(19.2172553122688,21.2721048743729,-8.94033126868766));
#95914=CARTESIAN_POINT('Ctrl Pts',(19.2881824098891,21.2554750089377,-8.94470504040463));
#95915=CARTESIAN_POINT('Ctrl Pts',(19.3583019532977,21.2351676251633,-8.9490788121216));
#95916=CARTESIAN_POINT('Ctrl Pts',(19.427209418299,21.211287404945,-8.95345258383858));
#95917=CARTESIAN_POINT('Ctrl Pts',(19.4960959145273,21.1874144515579,-8.95782502460213));
#95918=CARTESIAN_POINT('Ctrl Pts',(19.5637706090987,21.159970978065,-8.96219746536568));
#95919=CARTESIAN_POINT('Ctrl Pts',(19.6298449292373,21.1291112748639,-8.96656990612923));
#95920=CARTESIAN_POINT('Ctrl Pts',(19.6959209389035,21.0982507825767,-8.97094245869657));
#95921=CARTESIAN_POINT('Ctrl Pts',(19.7603960566779,21.0639740930878,-8.97531501126391));
#95922=CARTESIAN_POINT('Ctrl Pts',(19.8229039996995,21.0264826023508,-8.97968756383126));
#95923=CARTESIAN_POINT('Ctrl Pts',(19.8854768158221,20.9889522015306,-8.98406465439858));
#95924=CARTESIAN_POINT('Ctrl Pts',(19.9460779664243,20.9482005866786,-8.9884417449659));
#95925=CARTESIAN_POINT('Ctrl Pts',(20.0043687218628,20.9044734454702,-8.99281883553323));
#95926=CARTESIAN_POINT('Ctrl Pts',(20.0626913120462,20.8607224232471,-8.99719831659217));
#95927=CARTESIAN_POINT('Ctrl Pts',(20.1187006241989,20.8139929484578,-9.00157779765111));
#95928=CARTESIAN_POINT('Ctrl Pts',(20.1720918257197,20.7645703720135,-9.00595727871005));
#95929=CARTESIAN_POINT('Ctrl Pts',(20.2255776627869,20.7150601943841,-9.01034452236977));
#95930=CARTESIAN_POINT('Ctrl Pts',(20.2764357852875,20.662847728454,-9.01473176602948));
#95931=CARTESIAN_POINT('Ctrl Pts',(20.324399377934,20.608254027966,-9.0191190096892));
#95932=CARTESIAN_POINT('Ctrl Pts',(20.357009999173,20.5711355722704,-9.02210191262404));
#95933=CARTESIAN_POINT('Ctrl Pts',(20.3882834007584,20.5329170566125,-9.02508481555887));
#95934=CARTESIAN_POINT('Ctrl Pts',(20.4181471898432,20.4937069980878,-9.0280677184937));
#95935=CARTESIAN_POINT('Ctrl Pts',(20.4620804149045,20.4360242867296,-9.0324559274246));
#95936=CARTESIAN_POINT('Ctrl Pts',(20.5031324849612,20.3759692727541,-9.0368441363555));
#95937=CARTESIAN_POINT('Ctrl Pts',(20.541037663595,20.3138616787018,-9.0412323452864));
#95938=CARTESIAN_POINT('Ctrl Pts',(20.578886584659,20.2518462626167,-9.04561404138767));
#95939=CARTESIAN_POINT('Ctrl Pts',(20.6135976366774,20.1877847222598,-9.04999573748893));
#95940=CARTESIAN_POINT('Ctrl Pts',(20.6449465138839,20.1220282218873,-9.0543774335902));
#95941=CARTESIAN_POINT('Ctrl Pts',(20.6762585536648,20.0563489906358,-9.05875398084984));
#95942=CARTESIAN_POINT('Ctrl Pts',(20.7042160604134,19.9889791891847,-9.06313052810949));
#95943=CARTESIAN_POINT('Ctrl Pts',(20.7286399572991,19.9202957357449,-9.06750707536913));
#95944=CARTESIAN_POINT('Ctrl Pts',(20.7530483649043,19.851655840353,-9.0718808470861));
#95945=CARTESIAN_POINT('Ctrl Pts',(20.773927447788,19.7817043993275,-9.07625461880308));
#95946=CARTESIAN_POINT('Ctrl Pts',(20.7911462655829,19.7108382158241,-9.08062839052005));
#95947=CARTESIAN_POINT('Ctrl Pts',(20.8083598436338,19.6399935971384,-9.08500083128361));
#95948=CARTESIAN_POINT('Ctrl Pts',(20.8219152540694,19.5682352570614,-9.08937327204716));
#95949=CARTESIAN_POINT('Ctrl Pts',(20.8317319036236,19.4959734382704,-9.09374571281071));
#95950=CARTESIAN_POINT('Ctrl Pts',(20.8415488041906,19.4237097717368,-9.09811826537806));
#95951=CARTESIAN_POINT('Ctrl Pts',(20.847626691118,19.3509430791855,-9.10249081794541));
#95952=CARTESIAN_POINT('Ctrl Pts',(20.8499366445659,19.2780903583472,-9.10686337051275));
#95953=CARTESIAN_POINT('Ctrl Pts',(20.8522489953706,19.2051620282073,-9.11124046108008));
#95954=CARTESIAN_POINT('Ctrl Pts',(20.8507855897922,19.1321479746869,-9.11561755164741));
#95955=CARTESIAN_POINT('Ctrl Pts',(20.8455696643532,19.0594660018899,-9.11999464221474));
#95956=CARTESIAN_POINT('Ctrl Pts',(20.8403508903038,18.9867443347699,-9.12437412327368));
#95957=CARTESIAN_POINT('Ctrl Pts',(20.8313755754733,18.9143555885064,-9.12875360433262));
#95958=CARTESIAN_POINT('Ctrl Pts',(20.8187186547148,18.8427105341121,-9.13313308539157));
#95959=CARTESIAN_POINT('Ctrl Pts',(20.8060392996493,18.7709384893398,-9.13752032905129));
#95960=CARTESIAN_POINT('Ctrl Pts',(20.7896654157129,18.6999132392689,-9.14190757271102));
#95961=CARTESIAN_POINT('Ctrl Pts',(20.7697225362409,18.6300329136336,-9.14629481637074));
#95962=CARTESIAN_POINT('Ctrl Pts',(20.7561632998913,18.582521025854,-9.14927771930554));
#95963=CARTESIAN_POINT('Ctrl Pts',(20.7409552755656,18.53553808659,-9.15226062224034));
#95964=CARTESIAN_POINT('Ctrl Pts',(20.7241505240927,18.4892037050155,-9.15524352517514));
#95965=CARTESIAN_POINT('Ctrl Pts',(20.6994287137937,18.4210402577035,-9.15963173410604));
#95966=CARTESIAN_POINT('Ctrl Pts',(20.6711526578599,18.3540153233853,-9.16401994303694));
#95967=CARTESIAN_POINT('Ctrl Pts',(20.6394473542677,18.288525404082,-9.16840815196783));
#95968=CARTESIAN_POINT('Ctrl Pts',(20.6077891066029,18.2231326826774,-9.1727898480691));
#95969=CARTESIAN_POINT('Ctrl Pts',(20.5727119232317,18.159270884301,-9.17717154417036));
#95970=CARTESIAN_POINT('Ctrl Pts',(20.5343896652636,18.0973186931568,-9.18155324027163));
#95971=CARTESIAN_POINT('Ctrl Pts',(20.4961124389984,18.0354393007675,-9.18592978753126));
#95972=CARTESIAN_POINT('Ctrl Pts',(20.4545979656273,17.9754654662072,-9.19030633479091));
#95973=CARTESIAN_POINT('Ctrl Pts',(20.410066242825,17.9177517834296,-9.19468288205054));
#95974=CARTESIAN_POINT('Ctrl Pts',(20.365562761394,17.8600747018308,-9.19905665376752));
#95975=CARTESIAN_POINT('Ctrl Pts',(20.3180461211089,17.8046553090191,-9.20343042548449));
#95976=CARTESIAN_POINT('Ctrl Pts',(20.267779095091,17.7518184871436,-9.20780419720146));
#95977=CARTESIAN_POINT('Ctrl Pts',(20.2175273654979,17.6989977436906,-9.21217663796501));
#95978=CARTESIAN_POINT('Ctrl Pts',(20.1645272440668,17.6487583602253,-9.21654907872856));
#95979=CARTESIAN_POINT('Ctrl Pts',(20.1090800563606,17.6013901595109,-9.22092151949211));
#95980=CARTESIAN_POINT('Ctrl Pts',(20.0536314508637,17.5540207475865,-9.22529407205946));
#95981=CARTESIAN_POINT('Ctrl Pts',(19.9957360229245,17.5095229759785,-9.2296666246268));
#95982=CARTESIAN_POINT('Ctrl Pts',(19.9357287478822,17.4681468746582,-9.23403917719414));
#95983=CARTESIAN_POINT('Ctrl Pts',(19.8756591950264,17.4267278316594,-9.23841626776147));
#95984=CARTESIAN_POINT('Ctrl Pts',(19.8134738170563,17.3884372018123,-9.24279335832879));
#95985=CARTESIAN_POINT('Ctrl Pts',(19.7495364985934,17.353481596316,-9.24717044889612));
#95986=CARTESIAN_POINT('Ctrl Pts',(19.6855642615878,17.3185069002662,-9.25154992995506));
#95987=CARTESIAN_POINT('Ctrl Pts',(19.6198386140603,17.286871064273,-9.255929411014));
#95988=CARTESIAN_POINT('Ctrl Pts',(19.5527455102414,17.258733422542,-9.26030889207294));
#95989=CARTESIAN_POINT('Ctrl Pts',(19.4855334843462,17.2305459070299,-9.26469613573266));
#95990=CARTESIAN_POINT('Ctrl Pts',(19.4169496162066,17.2058691314341,-9.26908337939238));
#95991=CARTESIAN_POINT('Ctrl Pts',(19.3473966187371,17.1848130421597,-9.2734706230521));
#95992=CARTESIAN_POINT('Ctrl Pts',(19.3001072825685,17.1704969304131,-9.27645352598692));
#95993=CARTESIAN_POINT('Ctrl Pts',(19.252370250734,17.1578534982272,-9.27943642892174));
#95994=CARTESIAN_POINT('Ctrl Pts',(19.2043142751594,17.1469037128609,-9.28241933185657));
#95995=CARTESIAN_POINT('Ctrl Pts',(19.1336181560408,17.1307952618032,-9.28680754078746));
#95996=CARTESIAN_POINT('Ctrl Pts',(19.0619555004259,17.1182916243426,-9.29119574971836));
#95997=CARTESIAN_POINT('Ctrl Pts',(18.9897273628004,17.1095023159863,-9.29558395864926));
#95998=CARTESIAN_POINT('Ctrl Pts',(18.9176064237069,17.1007260524208,-9.29996565475052));
#95999=CARTESIAN_POINT('Ctrl Pts',(18.8449221435536,17.0956532323251,-9.30434735085179));
#96000=CARTESIAN_POINT('Ctrl Pts',(18.7720870435491,17.0943426405973,-9.30872904695306));
#96001=CARTESIAN_POINT('Ctrl Pts',(18.6993375305835,17.0930335889191,-9.3131055942127));
#96002=CARTESIAN_POINT('Ctrl Pts',(18.6264380297319,17.0954779920626,-9.31748214147234));
#96003=CARTESIAN_POINT('Ctrl Pts',(18.5538057789622,17.1016828017805,-9.32185868873197));
#96004=CARTESIAN_POINT('Ctrl Pts',(18.4812195905104,17.1078836764983,-9.32623246044895));
#96005=CARTESIAN_POINT('Ctrl Pts',(18.4089007953029,17.1178401850896,-9.33060623216592));
#96006=CARTESIAN_POINT('Ctrl Pts',(18.3372648019201,17.1315072294897,-9.33498000388289));
#96007=CARTESIAN_POINT('Ctrl Pts',(18.2656506076106,17.1451701149624,-9.33935244464644));
#96008=CARTESIAN_POINT('Ctrl Pts',(18.1947192761673,17.1625412042304,-9.34372488540999));
#96009=CARTESIAN_POINT('Ctrl Pts',(18.1248776044805,17.1835240057459,-9.34809732617354));
#96010=CARTESIAN_POINT('Ctrl Pts',(18.0550341469345,17.204507343794,-9.35246987874089));
#96011=CARTESIAN_POINT('Ctrl Pts',(17.9862808658674,17.2291024367364,-9.35684243130823));
#96012=CARTESIAN_POINT('Ctrl Pts',(17.9190093127146,17.257162959805,-9.36121498387557));
#96013=CARTESIAN_POINT('Ctrl Pts',(17.8516679426066,17.2852526051428,-9.3655920744429));
#96014=CARTESIAN_POINT('Ctrl Pts',(17.7858118168726,17.3168146752692,-9.36996916501022));
#96015=CARTESIAN_POINT('Ctrl Pts',(17.7218116266779,17.3516550355269,-9.37434625557755));
#96016=CARTESIAN_POINT('Ctrl Pts',(17.6577764836039,17.3865144233984,-9.37872573663649));
#96017=CARTESIAN_POINT('Ctrl Pts',(17.5955997055921,17.4246554136578,-9.38310521769543));
#96018=CARTESIAN_POINT('Ctrl Pts',(17.5356241771988,17.4658397244592,-9.38748469875437));
#96019=CARTESIAN_POINT('Ctrl Pts',(17.4755423425841,17.5070970341751,-9.39187194241409));
#96020=CARTESIAN_POINT('Ctrl Pts',(17.4176699324644,17.5514081430501,-9.3962591860738));
#96021=CARTESIAN_POINT('Ctrl Pts',(17.3623173752297,17.5984939451576,-9.40064642973352));
#96022=CARTESIAN_POINT('Ctrl Pts',(17.3246829700697,17.6305077534137,-9.40362933266835));
#96023=CARTESIAN_POINT('Ctrl Pts',(17.2882126945403,17.6638033925969,-9.40661223560317));
#96024=CARTESIAN_POINT('Ctrl Pts',(17.2529938697635,17.6982839518925,-9.409595138538));
#96025=CARTESIAN_POINT('Ctrl Pts',(17.2019263404371,17.7482809913786,-9.4139203675616));
#96026=CARTESIAN_POINT('Ctrl Pts',(17.1532799906061,17.800978288147,-9.4182455965852));
#96027=CARTESIAN_POINT('Ctrl Pts',(17.1073599831677,17.8561083970887,-9.42257082560881));
#96028=CARTESIAN_POINT('Ctrl Pts',(17.0615168757445,17.9111461823036,-9.42688881138058));
#96029=CARTESIAN_POINT('Ctrl Pts',(17.0183913618817,17.9686083127059,-9.43120679715236));
#96030=CARTESIAN_POINT('Ctrl Pts',(16.9782524640738,18.0281899602688,-9.43552478292413));
#96031=CARTESIAN_POINT('Ctrl Pts',(16.9381523085285,18.0877140993308,-9.43983860095469));
#96032=CARTESIAN_POINT('Ctrl Pts',(16.90103333123,18.1493532901009,-9.44415241898526));
#96033=CARTESIAN_POINT('Ctrl Pts',(16.8671239501056,18.212770159567,-9.44846623701582));
#96034=CARTESIAN_POINT('Ctrl Pts',(16.8332351489704,18.2761485406136,-9.45277743694114));
#96035=CARTESIAN_POINT('Ctrl Pts',(16.8025523148359,18.3413020229706,-9.45708863686646));
#96036=CARTESIAN_POINT('Ctrl Pts',(16.775259218471,18.4078664178513,-9.46139983679178));
#96037=CARTESIAN_POINT('Ctrl Pts',(16.7648137942846,18.433341480517,-9.4630497892695));
#96038=CARTESIAN_POINT('Ctrl Pts',(16.7548643811019,18.459022946162,-9.46469974174723));
#96039=CARTESIAN_POINT('Ctrl Pts',(16.7454194503191,18.4848895418526,-9.46634969422496));
#96040=CARTESIAN_POINT('',(16.6170008950802,19.2129467328109,-8.48905627902251));
#96041=CARTESIAN_POINT('Ctrl Pts',(16.7454193052938,18.48488993903,-9.24346979856369));
#96042=CARTESIAN_POINT('Ctrl Pts',(16.7776919628128,18.3965055643205,-9.23734830228666));
#96043=CARTESIAN_POINT('Ctrl Pts',(16.8158509820645,18.3102897988965,-9.23135282458082));
#96044=CARTESIAN_POINT('Ctrl Pts',(16.8706991286688,18.205832638464,-9.22408567598336));
#96045=CARTESIAN_POINT('Ctrl Pts',(16.8820779852137,18.1850192571194,-9.22263707444487));
#96046=CARTESIAN_POINT('Ctrl Pts',(16.8985836792739,18.1559979252235,-9.22061560309788));
#96047=CARTESIAN_POINT('Ctrl Pts',(16.9034203259883,18.1476277650252,-9.2200323875879));
#96048=CARTESIAN_POINT('Ctrl Pts',(16.9113459932644,18.1341261735529,-9.2190912223094));
#96049=CARTESIAN_POINT('Ctrl Pts',(16.9143997135171,18.1289742771388,-9.21873199941962));
#96050=CARTESIAN_POINT('Ctrl Pts',(16.9208165120184,18.118252558687,-9.21798418250105));
#96051=CARTESIAN_POINT('Ctrl Pts',(16.9241834921427,18.1126851357967,-9.21759573585337));
#96052=CARTESIAN_POINT('Ctrl Pts',(16.9322157232303,18.0995407826206,-9.21667827751021));
#96053=CARTESIAN_POINT('Ctrl Pts',(16.9369032060674,18.0919775297912,-9.2161500884325));
#96054=CARTESIAN_POINT('Ctrl Pts',(16.9526728384797,18.0668878897934,-9.21439677833209));
#96055=CARTESIAN_POINT('Ctrl Pts',(16.9639650076356,18.0494944477354,-9.2131794334003));
#96056=CARTESIAN_POINT('Ctrl Pts',(17.025608981099,17.9575309212493,-9.20672828037623));
#96057=CARTESIAN_POINT('Ctrl Pts',(17.0804234607416,17.8860577695434,-9.20166743052635));
#96058=CARTESIAN_POINT('Ctrl Pts',(17.2287759526704,17.7162246665542,-9.18922997537975));
#96059=CARTESIAN_POINT('Ctrl Pts',(17.3275149905598,17.6229664971023,-9.18201737714853));
#96060=CARTESIAN_POINT('Ctrl Pts',(17.4939961859353,17.4935127703042,-9.17034166014399));
#96061=CARTESIAN_POINT('Ctrl Pts',(17.5559294866221,17.4504548711986,-9.16608160644238));
#96062=CARTESIAN_POINT('Ctrl Pts',(17.6280883177326,17.4058023925679,-9.16105237100025));
#96063=CARTESIAN_POINT('Ctrl Pts',(17.6361910981013,17.4008633592509,-9.16048672669509));
#96064=CARTESIAN_POINT('Ctrl Pts',(17.6482528121486,17.3936219394439,-9.15964295424813));
#96065=CARTESIAN_POINT('Ctrl Pts',(17.6521865813448,17.391277576873,-9.1593674935711));
#96066=CARTESIAN_POINT('Ctrl Pts',(17.6592019857842,17.3871274754381,-9.15887569647239));
#96067=CARTESIAN_POINT('Ctrl Pts',(17.6622806146186,17.3853167536561,-9.15865968854461));
#96068=CARTESIAN_POINT('Ctrl Pts',(17.6689127366999,17.3814385709335,-9.15819393383801));
#96069=CARTESIAN_POINT('Ctrl Pts',(17.6724676221806,17.3793736976805,-9.15794403109686));
#96070=CARTESIAN_POINT('Ctrl Pts',(17.6823047346558,17.3736980178888,-9.15725184780603));
#96071=CARTESIAN_POINT('Ctrl Pts',(17.6885994512144,17.3701091304156,-9.15680819358444));
#96072=CARTESIAN_POINT('Ctrl Pts',(17.7233170773638,17.3505506122997,-9.15435780814619));
#96073=CARTESIAN_POINT('Ctrl Pts',(17.7520858943435,17.3352078172821,-9.15231458744777));
#96074=CARTESIAN_POINT('Ctrl Pts',(17.9264391570361,17.247332778966,-9.13990716426774));
#96075=CARTESIAN_POINT('Ctrl Pts',(18.0796306930682,17.1911128202525,-9.12895411249994));
#96076=CARTESIAN_POINT('Ctrl Pts',(18.3512845594647,17.1256083792614,-9.11070140886584));
#96077=CARTESIAN_POINT('Ctrl Pts',(18.4669069626635,17.107669680694,-9.10326189030197));
#96078=CARTESIAN_POINT('Ctrl Pts',(18.597689201516,17.0983446698309,-9.09525606336226));
#96079=CARTESIAN_POINT('Ctrl Pts',(18.6119522884755,17.0974727232176,-9.09438810351552));
#96080=CARTESIAN_POINT('Ctrl Pts',(18.6346668635054,17.0963148211881,-9.09301381567209));
#96081=CARTESIAN_POINT('Ctrl Pts',(18.6431129328172,17.0959349840369,-9.09250455974448));
#96082=CARTESIAN_POINT('Ctrl Pts',(18.6580129557076,17.0953543164926,-9.09160918708027));
#96083=CARTESIAN_POINT('Ctrl Pts',(18.6644659347314,17.0951323991696,-9.0912224142415));
#96084=CARTESIAN_POINT('Ctrl Pts',(18.6778149088786,17.0947344639315,-9.09042434454801));
#96085=CARTESIAN_POINT('Ctrl Pts',(18.6847109589082,17.0945626218158,-9.09001318308699));
#96086=CARTESIAN_POINT('Ctrl Pts',(18.7024144115813,17.0942080450498,-9.08896046344141));
#96087=CARTESIAN_POINT('Ctrl Pts',(18.7132226811078,17.0940743660874,-9.08832044661547));
#96088=CARTESIAN_POINT('Ctrl Pts',(18.758337611066,17.0938619304738,-9.08565970298393));
#96089=CARTESIAN_POINT('Ctrl Pts',(18.7926437396989,17.0945343061688,-9.08366250668527));
#96090=CARTESIAN_POINT('Ctrl Pts',(18.8819744299117,17.0984590128382,-9.07851821364631));
#96091=CARTESIAN_POINT('Ctrl Pts',(18.9369160423201,17.1030266653512,-9.07541051022945));
#96092=CARTESIAN_POINT('Ctrl Pts',(19.1001558859863,17.1230402340134,-9.06626584779699));
#96093=CARTESIAN_POINT('Ctrl Pts',(19.2075006637055,17.1447366764978,-9.06037761733385));
#96094=CARTESIAN_POINT('Ctrl Pts',(19.3568853721499,17.187188268377,-9.05192245191781));
#96095=CARTESIAN_POINT('Ctrl Pts',(19.4006604436814,17.2011831617325,-9.04941012011181));
#96096=CARTESIAN_POINT('Ctrl Pts',(19.4649345943963,17.2240626462079,-9.04562649873492));
#96097=CARTESIAN_POINT('Ctrl Pts',(19.4858052914449,17.2318652939893,-9.04438267659672));
#96098=CARTESIAN_POINT('Ctrl Pts',(19.5544072084081,17.2587542776347,-9.04023203251112));
#96099=CARTESIAN_POINT('Ctrl Pts',(19.6015628117564,17.2792481541047,-9.03727832061984));
#96100=CARTESIAN_POINT('Ctrl Pts',(19.6550272041254,17.3048363284226,-9.03376033661468));
#96101=CARTESIAN_POINT('Ctrl Pts',(19.6621135787784,17.3082766270149,-9.03329054303779));
#96102=CARTESIAN_POINT('Ctrl Pts',(19.6733812409581,17.3138247816437,-9.03253768488937));
#96103=CARTESIAN_POINT('Ctrl Pts',(19.6775750985913,17.3159071375355,-9.03225616553865));
#96104=CARTESIAN_POINT('Ctrl Pts',(19.6849748705664,17.3196119631652,-9.0317570766856));
#96105=CARTESIAN_POINT('Ctrl Pts',(19.6881836056666,17.3212287025002,-9.0315398671278));
#96106=CARTESIAN_POINT('Ctrl Pts',(19.6949586638533,17.3246640088137,-9.03107954395319));
#96107=CARTESIAN_POINT('Ctrl Pts',(19.6985238934903,17.3264844963357,-9.03083631546905));
#96108=CARTESIAN_POINT('Ctrl Pts',(19.7080942453642,17.3314056084365,-9.03018077323934));
#96109=CARTESIAN_POINT('Ctrl Pts',(19.7140896595904,17.3345248650829,-9.02976731167012));
#96110=CARTESIAN_POINT('Ctrl Pts',(19.743292562101,17.349896500763,-9.02774010467501));
#96111=CARTESIAN_POINT('Ctrl Pts',(19.7662846696949,17.3625503996603,-9.02610291813721));
#96112=CARTESIAN_POINT('Ctrl Pts',(19.8314668289078,17.4000193195941,-9.02135529847618));
#96113=CARTESIAN_POINT('Ctrl Pts',(19.8730379760785,17.4258735837705,-9.01819730213773));
#96114=CARTESIAN_POINT('Ctrl Pts',(19.9939287975699,17.5070017119041,-9.00869692007588));
#96115=CARTESIAN_POINT('Ctrl Pts',(20.0704010149636,17.5662924672909,-9.00226770257484));
#96116=CARTESIAN_POINT('Ctrl Pts',(20.2478288301528,17.7244275561139,-8.98663169643754));
#96117=CARTESIAN_POINT('Ctrl Pts',(20.3434811724073,17.8285532324758,-8.97756398980603));
#96118=CARTESIAN_POINT('Ctrl Pts',(20.4366435887765,17.9528673372903,-8.96807848916196));
#96119=CARTESIAN_POINT('Ctrl Pts',(20.4450930116034,17.9643830946458,-8.96721093976882));
#96120=CARTESIAN_POINT('Ctrl Pts',(20.458356437897,17.9828488204215,-8.96583717693133));
#96121=CARTESIAN_POINT('Ctrl Pts',(20.4632463580122,17.989743482574,-8.96532803903539));
#96122=CARTESIAN_POINT('Ctrl Pts',(20.4717983596235,18.0019559370133,-8.96443280365217));
#96123=CARTESIAN_POINT('Ctrl Pts',(20.4754776279023,18.0072615076762,-8.96404605069599));
#96124=CARTESIAN_POINT('Ctrl Pts',(20.4830379938458,18.0182709064741,-8.9632479547465));
#96125=CARTESIAN_POINT('Ctrl Pts',(20.486915601317,18.0239770470414,-8.96283674747862));
#96126=CARTESIAN_POINT('Ctrl Pts',(20.4967986448851,18.0386745993831,-8.96178377123622));
#96127=CARTESIAN_POINT('Ctrl Pts',(20.502763262808,18.0476933190054,-8.96114354509566));
#96128=CARTESIAN_POINT('Ctrl Pts',(20.5273802987274,18.0855422402812,-8.95848076621297));
#96129=CARTESIAN_POINT('Ctrl Pts',(20.5453996095743,18.1147793486944,-8.95648178994889));
#96130=CARTESIAN_POINT('Ctrl Pts',(20.5904987855703,18.1921056400121,-8.95133187489823));
#96131=CARTESIAN_POINT('Ctrl Pts',(20.6164243500648,18.2408388425351,-8.94822044244671));
#96132=CARTESIAN_POINT('Ctrl Pts',(20.6879870350135,18.389055174631,-8.93906927501836));
#96133=CARTESIAN_POINT('Ctrl Pts',(20.7278486872358,18.491120205809,-8.9331782467684));
#96134=CARTESIAN_POINT('Ctrl Pts',(20.7744406658072,18.6445337473782,-8.92444876472104));
#96135=CARTESIAN_POINT('Ctrl Pts',(20.7874752342794,18.693775446934,-8.92166302191361));
#96136=CARTESIAN_POINT('Ctrl Pts',(20.8021904349712,18.7587566567361,-8.9179561528775));
#96137=CARTESIAN_POINT('Ctrl Pts',(20.8054888854613,18.7741138627915,-8.91707785508989));
#96138=CARTESIAN_POINT('Ctrl Pts',(20.8191178673619,18.8411964544295,-8.91322621911917));
#96139=CARTESIAN_POINT('Ctrl Pts',(20.8276832239092,18.893256782039,-8.91019826495504));
#96140=CARTESIAN_POINT('Ctrl Pts',(20.8353850229947,18.9542013615242,-8.90655266399877));
#96141=CARTESIAN_POINT('Ctrl Pts',(20.836421686787,18.9628315075318,-8.90603407798051));
#96142=CARTESIAN_POINT('Ctrl Pts',(20.8379117366309,18.9759160791536,-8.90524394387023));
#96143=CARTESIAN_POINT('Ctrl Pts',(20.838404200869,18.9803660825203,-8.90497454360295));
#96144=CARTESIAN_POINT('Ctrl Pts',(20.8392632772284,18.9883607565961,-8.90448927829947));
#96145=CARTESIAN_POINT('Ctrl Pts',(20.8396350585575,18.9919048174373,-8.90427370731551));
#96146=CARTESIAN_POINT('Ctrl Pts',(20.8404239564097,18.9996126160795,-8.90380387986917));
#96147=CARTESIAN_POINT('Ctrl Pts',(20.8408376712917,19.0037766028078,-8.90354944046532));
#96148=CARTESIAN_POINT('Ctrl Pts',(20.8419662918357,19.0154888736914,-8.90283206232885));
#96149=CARTESIAN_POINT('Ctrl Pts',(20.8426529866629,19.0230397226283,-8.90236758445281));
#96150=CARTESIAN_POINT('Ctrl Pts',(20.8465378364671,19.0684612085059,-8.89956227655246));
#96151=CARTESIAN_POINT('Ctrl Pts',(20.8487560454108,19.1064061638141,-8.89717169202978));
#96152=CARTESIAN_POINT('Ctrl Pts',(20.8527120497115,19.2320687438044,-8.88914350192847));
#96153=CARTESIAN_POINT('Ctrl Pts',(20.8500194721709,19.3198315215465,-8.88336090979676));
#96154=CARTESIAN_POINT('Ctrl Pts',(20.8257291667823,19.580839202345,-8.86604055281282));
#96155=CARTESIAN_POINT('Ctrl Pts',(20.7881616968977,19.7518832770795,-8.85459338990223));
#96156=CARTESIAN_POINT('Ctrl Pts',(20.7223353818401,19.9381474700761,-8.84243270707467));
#96157=CARTESIAN_POINT('Ctrl Pts',(20.7142945280051,19.9597687776114,-8.84102454826613));
#96158=CARTESIAN_POINT('Ctrl Pts',(20.7024238959517,19.9901583468403,-8.83904951872588));
#96159=CARTESIAN_POINT('Ctrl Pts',(20.6988858279249,19.99903810283,-8.83847292825812));
#96160=CARTESIAN_POINT('Ctrl Pts',(20.6930407961322,20.0134236963241,-8.83753957100816));
#96161=CARTESIAN_POINT('Ctrl Pts',(20.6907705021299,20.0189442013288,-8.83718157202157));
#96162=CARTESIAN_POINT('Ctrl Pts',(20.6859705804276,20.0304769045404,-8.83643403358372));
#96163=CARTESIAN_POINT('Ctrl Pts',(20.6834364511057,20.0364871704023,-8.83604465148605));
#96164=CARTESIAN_POINT('Ctrl Pts',(20.6773439851273,20.0507523192948,-8.83512088843328));
#96165=CARTESIAN_POINT('Ctrl Pts',(20.67376075126,20.0589964822795,-8.83458736156573));
#96166=CARTESIAN_POINT('Ctrl Pts',(20.6615229511862,20.0866692486636,-8.83279743471176));
#96167=CARTESIAN_POINT('Ctrl Pts',(20.6526279636924,20.1059905842415,-8.83154927045854));
#96168=CARTESIAN_POINT('Ctrl Pts',(20.5767424343973,20.2644931444036,-8.82131514099577));
#96169=CARTESIAN_POINT('Ctrl Pts',(20.4949943643222,20.396096532477,-8.81289769681896));
#96170=CARTESIAN_POINT('Ctrl Pts',(20.3152269098503,20.6252547001897,-8.79708100175859));
#96171=CARTESIAN_POINT('Ctrl Pts',(20.2205925139279,20.7244157436544,-8.78969554797914));
#96172=CARTESIAN_POINT('Ctrl Pts',(20.1052750743133,20.8239279618765,-8.78076350901784));
#96173=CARTESIAN_POINT('Ctrl Pts',(20.0933630696947,20.8339799605896,-8.77984139888985));
#96174=CARTESIAN_POINT('Ctrl Pts',(20.0768874881666,20.8475743305974,-8.77856504034232));
#96175=CARTESIAN_POINT('Ctrl Pts',(20.0724184618654,20.8512311924251,-8.77821872873846));
#96176=CARTESIAN_POINT('Ctrl Pts',(20.0652882320271,20.8570170891768,-8.77766594018967));
#96177=CARTESIAN_POINT('Ctrl Pts',(20.062636714158,20.859158091934,-8.77746031881893));
#96178=CARTESIAN_POINT('Ctrl Pts',(20.0571456323476,20.8635700760263,-8.77703435075884));
#96179=CARTESIAN_POINT('Ctrl Pts',(20.0543053918273,20.8658401409539,-8.77681393885086));
#96180=CARTESIAN_POINT('Ctrl Pts',(20.0475167831172,20.8712373412698,-8.77628695102302));
#96181=CARTESIAN_POINT('Ctrl Pts',(20.0435630875839,20.8743577147781,-8.77597989750151));
#96182=CARTESIAN_POINT('Ctrl Pts',(20.0301589877917,20.8848592145884,-8.77493855717006));
#96183=CARTESIAN_POINT('Ctrl Pts',(20.0206572188367,20.8921739879757,-8.77419980455329));
#96184=CARTESIAN_POINT('Ctrl Pts',(19.909385762269,20.9763385764823,-8.76554692061459));
#96185=CARTESIAN_POINT('Ctrl Pts',(19.8009445826786,21.0439142080287,-8.75711384414727));
#96186=CARTESIAN_POINT('Ctrl Pts',(19.5397082052372,21.1756295451071,-8.73778005157247));
#96187=CARTESIAN_POINT('Ctrl Pts',(19.3841059672341,21.2324640429033,-8.72698432156367));
#96188=CARTESIAN_POINT('Ctrl Pts',(19.2004907617823,21.2760986884311,-8.71536072834314));
#96189=CARTESIAN_POINT('Ctrl Pts',(19.1774343868463,21.281172031292,-8.71391912030088));
#96190=CARTESIAN_POINT('Ctrl Pts',(19.144841289946,21.2877743060172,-8.71190568615215));
#96191=CARTESIAN_POINT('Ctrl Pts',(19.1353722527908,21.289625123289,-8.71132362378549));
#96192=CARTESIAN_POINT('Ctrl Pts',(19.1200088330267,21.292519158126,-8.71038381860314));
#96193=CARTESIAN_POINT('Ctrl Pts',(19.1141221777934,21.2936022077952,-8.71002480981884));
#96194=CARTESIAN_POINT('Ctrl Pts',(19.1018244546276,21.2958109117717,-8.70927704807292));
#96195=CARTESIAN_POINT('Ctrl Pts',(19.0954126212641,21.2969319945566,-8.70888844420598));
#96196=CARTESIAN_POINT('Ctrl Pts',(19.0802085171673,21.2995181614255,-8.70796991567415));
#96197=CARTESIAN_POINT('Ctrl Pts',(19.0714119184816,21.3009573318447,-8.70744081896162));
#96198=CARTESIAN_POINT('Ctrl Pts',(19.0426186901461,21.3054815290722,-8.70571639971669));
#96199=CARTESIAN_POINT('Ctrl Pts',(19.0225865079875,21.3083355098344,-8.70452838897926));
#96200=CARTESIAN_POINT('Ctrl Pts',(18.9749201705925,21.3144306384531,-8.70172734196657));
#96201=CARTESIAN_POINT('Ctrl Pts',(18.9472566684265,21.3174151236312,-8.70012226493225));
#96202=CARTESIAN_POINT('Ctrl Pts',(18.7508332121769,21.3346968790879,-8.68885156679276));
#96203=CARTESIAN_POINT('Ctrl Pts',(18.5809587337328,21.3292428538322,-8.67982437037039));
#96204=CARTESIAN_POINT('Ctrl Pts',(18.3107879914595,21.287869456652,-8.66488754094842));
#96205=CARTESIAN_POINT('Ctrl Pts',(18.2093450688665,21.264588689951,-8.65912326933674));
#96206=CARTESIAN_POINT('Ctrl Pts',(18.1007796334846,21.2311026760289,-8.65239231796164));
#96207=CARTESIAN_POINT('Ctrl Pts',(18.0915420559092,21.2281838380001,-8.65181500571073));
#96208=CARTESIAN_POINT('Ctrl Pts',(18.0779311510278,21.2237801649908,-8.65095713719026));
#96209=CARTESIAN_POINT('Ctrl Pts',(18.0735419765791,21.2223442086189,-8.65067937941425));
#96210=CARTESIAN_POINT('Ctrl Pts',(18.0657629051375,21.2197710098002,-8.65018505905114));
#96211=CARTESIAN_POINT('Ctrl Pts',(18.0623711538575,21.2186395287958,-8.64996883797312));
#96212=CARTESIAN_POINT('Ctrl Pts',(18.055109491007,21.2161965919531,-8.64950441099816));
#96213=CARTESIAN_POINT('Ctrl Pts',(18.0512405633225,21.2148825431039,-8.64925605851655));
#96214=CARTESIAN_POINT('Ctrl Pts',(18.0406289361819,21.211244093855,-8.64857242500047));
#96215=CARTESIAN_POINT('Ctrl Pts',(18.0338942132641,21.2088968319668,-8.6481358245441));
#96216=CARTESIAN_POINT('Ctrl Pts',(17.9984775022011,21.1963519351799,-8.64582590217721));
#96217=CARTESIAN_POINT('Ctrl Pts',(17.9700076541501,21.1855711240172,-8.64392087772381));
#96218=CARTESIAN_POINT('Ctrl Pts',(17.791421086757,21.1135046606052,-8.63170745357483));
#96219=CARTESIAN_POINT('Ctrl Pts',(17.6485335709652,21.035757754653,-8.62079146716301));
#96220=CARTESIAN_POINT('Ctrl Pts',(17.4180930384394,20.8736439229559,-8.60236920622934));
#96221=CARTESIAN_POINT('Ctrl Pts',(17.3262604550972,20.7966461369471,-8.59474158559478));
#96222=CARTESIAN_POINT('Ctrl Pts',(17.230271194464,20.7012132334795,-8.58647639043208));
#96223=CARTESIAN_POINT('Ctrl Pts',(17.2192537691211,20.6900130759247,-8.58552258377925));
#96224=CARTESIAN_POINT('Ctrl Pts',(17.2027731923036,20.6728818158145,-8.5840876559297));
#96225=CARTESIAN_POINT('Ctrl Pts',(17.1972177502904,20.6670406243646,-8.58360251809225));
#96226=CARTESIAN_POINT('Ctrl Pts',(17.1873222629956,20.6565164268532,-8.58273572869331));
#96227=CARTESIAN_POINT('Ctrl Pts',(17.1829698066778,20.6518452738702,-8.58235354445013));
#96228=CARTESIAN_POINT('Ctrl Pts',(17.1737790492117,20.6418916438198,-8.58154448539988));
#96229=CARTESIAN_POINT('Ctrl Pts',(17.1689462846402,20.6366041461803,-8.58111784938631));
#96230=CARTESIAN_POINT('Ctrl Pts',(17.1591629009864,20.6257904988035,-8.58025163899237));
#96231=CARTESIAN_POINT('Ctrl Pts',(17.1542143061841,20.6202626468025,-8.57981215285311));
#96232=CARTESIAN_POINT('Ctrl Pts',(17.1324256586633,20.5956645382183,-8.57787095880103));
#96233=CARTESIAN_POINT('Ctrl Pts',(17.1159006587748,20.5763171273516,-8.57638235707686));
#96234=CARTESIAN_POINT('Ctrl Pts',(17.0457286186244,20.4910958580706,-8.56998123679427));
#96235=CARTESIAN_POINT('Ctrl Pts',(16.9957224886823,20.4223212459699,-8.56521401257862));
#96236=CARTESIAN_POINT('Ctrl Pts',(16.9128101519597,20.2925375766098,-8.55672636591948));
#96237=CARTESIAN_POINT('Ctrl Pts',(16.8785074356792,20.2325692289229,-8.55298123514122));
#96238=CARTESIAN_POINT('Ctrl Pts',(16.7878577128624,20.0544101491626,-8.54212537198846));
#96239=CARTESIAN_POINT('Ctrl Pts',(16.7394673000962,19.9325542232887,-8.53503483658883));
#96240=CARTESIAN_POINT('Ctrl Pts',(16.6982006722433,19.7919117099035,-8.52644200519389));
#96241=CARTESIAN_POINT('Ctrl Pts',(16.6939331602703,19.7767424980478,-8.52550991017736));
#96242=CARTESIAN_POINT('Ctrl Pts',(16.6883270785654,19.7559265504045,-8.52422183517333));
#96243=CARTESIAN_POINT('Ctrl Pts',(16.6868416776121,19.7503194304885,-8.52387398124809));
#96244=CARTESIAN_POINT('Ctrl Pts',(16.6845188928791,19.7414034699987,-8.52331933924958));
#96245=CARTESIAN_POINT('Ctrl Pts',(16.6836664224201,19.7380985388894,-8.52311341706873));
#96246=CARTESIAN_POINT('Ctrl Pts',(16.681923128137,19.7312717645712,-8.52268734978282));
#96247=CARTESIAN_POINT('Ctrl Pts',(16.6810333787433,19.7277496959568,-8.5224671418051));
#96248=CARTESIAN_POINT('Ctrl Pts',(16.6789361653896,19.7193569780708,-8.5219415020895));
#96249=CARTESIAN_POINT('Ctrl Pts',(16.677736949469,19.7144843069132,-8.52163559917055));
#96250=CARTESIAN_POINT('Ctrl Pts',(16.6752325974941,19.70415039399,-8.52098537573012));
#96251=CARTESIAN_POINT('Ctrl Pts',(16.6739318448009,19.6986881411743,-8.52064081713856));
#96252=CARTESIAN_POINT('Ctrl Pts',(16.6704195264811,19.6836740509122,-8.51969147471348));
#96253=CARTESIAN_POINT('Ctrl Pts',(16.6682525933811,19.6741120524001,-8.51908436795847));
#96254=CARTESIAN_POINT('Ctrl Pts',(16.6336164633659,19.5161922485616,-8.50902048576369));
#96255=CARTESIAN_POINT('Ctrl Pts',(16.6171414698285,19.3647964194431,-8.49886432390527));
#96256=CARTESIAN_POINT('Ctrl Pts',(16.617000907147,19.2129598110916,-8.48885784168996));
#96257=CARTESIAN_POINT('Ctrl Pts',(16.6170008950802,19.2129467328109,-8.48905627902251));
#96258=CARTESIAN_POINT('Ctrl Pts',(16.6169347305481,19.1409952794385,-8.48473008583425));
#96259=CARTESIAN_POINT('Ctrl Pts',(16.6205409900205,19.0689489014299,-8.480403892646));
#96260=CARTESIAN_POINT('Ctrl Pts',(16.6278220014955,18.9972168420672,-8.47607769945775));
#96261=CARTESIAN_POINT('Ctrl Pts',(16.6350980157525,18.9255340149771,-8.47175447549028));
#96262=CARTESIAN_POINT('Ctrl Pts',(16.6460437282405,18.8541655692476,-8.46743125152281));
#96263=CARTESIAN_POINT('Ctrl Pts',(16.6606094541867,18.7835182523991,-8.46310802755535));
#96264=CARTESIAN_POINT('Ctrl Pts',(16.6751723924898,18.712884456298,-8.45878563098263));
#96265=CARTESIAN_POINT('Ctrl Pts',(16.6933538757663,18.6429720006072,-8.45446323440992));
#96266=CARTESIAN_POINT('Ctrl Pts',(16.715052943236,18.5741783750656,-8.4501408378372));
#96267=CARTESIAN_POINT('Ctrl Pts',(16.7245112167564,18.5441923432816,-8.44825677488816));
#96268=CARTESIAN_POINT('Ctrl Pts',(16.7346371624495,18.5144187239461,-8.44637271193913));
#96269=CARTESIAN_POINT('Ctrl Pts',(16.7454194503191,18.4848895418526,-8.44448864899009));
#96270=CARTESIAN_POINT('Origin',(18.734,19.211,0.));
#96271=CARTESIAN_POINT('',(16.743090251011,18.4840590306076,-7.64456001983877));
#96272=CARTESIAN_POINT('',(16.7454194594376,18.48488951688,-7.86510585860832));
#96273=CARTESIAN_POINT('',(16.7454194503191,18.4848895418526,0.));
#96274=CARTESIAN_POINT('Ctrl Pts',(16.7454194594376,18.48488951688,-7.86510585860832));
#96275=CARTESIAN_POINT('Ctrl Pts',(16.7304230273875,18.5259598686323,-7.86752223947087));
#96276=CARTESIAN_POINT('Ctrl Pts',(16.7166995325181,18.5674931908287,-7.86996740497596));
#96277=CARTESIAN_POINT('Ctrl Pts',(16.6934926739549,18.6457943982049,-7.87462968920152));
#96278=CARTESIAN_POINT('Ctrl Pts',(16.6836949825475,18.6824392626494,-7.87683263687354));
#96279=CARTESIAN_POINT('Ctrl Pts',(16.6731275207629,18.7266952968784,-7.87953974144989));
#96280=CARTESIAN_POINT('Ctrl Pts',(16.6714072151537,18.7340750361865,-7.87999269565253));
#96281=CARTESIAN_POINT('Ctrl Pts',(16.6687987096677,18.7455430926281,-7.8806991972288));
#96282=CARTESIAN_POINT('Ctrl Pts',(16.6678829269928,18.7496251609123,-7.8809511901207));
#96283=CARTESIAN_POINT('Ctrl Pts',(16.6662094739841,18.7571894224134,-7.88141913869248));
#96284=CARTESIAN_POINT('Ctrl Pts',(16.6654484940501,18.7606708243268,-7.88163490202922));
#96285=CARTESIAN_POINT('Ctrl Pts',(16.6637510198014,18.7685316774695,-7.88212296858969));
#96286=CARTESIAN_POINT('Ctrl Pts',(16.6628196353636,18.7729121632044,-7.88239555828951));
#96287=CARTESIAN_POINT('Ctrl Pts',(16.6601202278895,18.7858090473554,-7.88319984325998));
#96288=CARTESIAN_POINT('Ctrl Pts',(16.6583908088322,18.7943333047062,-7.88373366240642));
#96289=CARTESIAN_POINT('Ctrl Pts',(16.6465062920967,18.85482238317,-7.88753626291812));
#96290=CARTESIAN_POINT('Ctrl Pts',(16.6382522074567,18.9071371206529,-7.89090068528666));
#96291=CARTESIAN_POINT('Ctrl Pts',(16.6301911627696,18.974565077764,-7.89528836083577));
#96292=CARTESIAN_POINT('Ctrl Pts',(16.6285719054459,18.9894472536599,-7.89625998535145));
#96293=CARTESIAN_POINT('Ctrl Pts',(16.6204362978251,19.0723914475444,-7.90168906101013));
#96294=CARTESIAN_POINT('Ctrl Pts',(16.6170625898628,19.1407193800489,-7.90621168660917));
#96295=CARTESIAN_POINT('Ctrl Pts',(16.6168557120902,19.3698585925268,-7.92135265286688));
#96296=CARTESIAN_POINT('Ctrl Pts',(16.6350247735365,19.530150830852,-7.93185065292163));
#96297=CARTESIAN_POINT('Ctrl Pts',(16.6765204029089,19.7100311479728,-7.94322215530368));
#96298=CARTESIAN_POINT('Ctrl Pts',(16.6822553139608,19.7331093704894,-7.94467443488116));
#96299=CARTESIAN_POINT('Ctrl Pts',(16.6908695969325,19.7654373693153,-7.94670013382866));
#96300=CARTESIAN_POINT('Ctrl Pts',(16.6934253009023,19.7747708246252,-7.94728395666081));
#96301=CARTESIAN_POINT('Ctrl Pts',(16.6976666647595,19.7898535532205,-7.94822583847425));
#96302=CARTESIAN_POINT('Ctrl Pts',(16.6993128688605,19.7956136910896,-7.94858517434873));
#96303=CARTESIAN_POINT('Ctrl Pts',(16.7027975181071,19.8076136024063,-7.9493330215632));
#96304=CARTESIAN_POINT('Ctrl Pts',(16.7046403188121,19.8138520538656,-7.9497213864207));
#96305=CARTESIAN_POINT('Ctrl Pts',(16.7090695326654,19.8285958470613,-7.95063828588326));
#96306=CARTESIAN_POINT('Ctrl Pts',(16.7116808365843,19.837093629421,-7.95116600065597));
#96307=CARTESIAN_POINT('Ctrl Pts',(16.7205471831887,19.8653124547349,-7.95291608286521));
#96308=CARTESIAN_POINT('Ctrl Pts',(16.7270379030043,19.8849586188442,-7.95413071405547));
#96309=CARTESIAN_POINT('Ctrl Pts',(16.7631661588376,19.9891582412885,-7.9605572763748));
#96310=CARTESIAN_POINT('Ctrl Pts',(16.7978624881053,20.0718661140701,-7.96559778768087));
#96311=CARTESIAN_POINT('Ctrl Pts',(16.8976428101316,20.2729144893916,-7.97797941932697));
#96312=CARTESIAN_POINT('Ctrl Pts',(16.9689850994329,20.3876861982128,-7.98515786453301));
#96313=CARTESIAN_POINT('Ctrl Pts',(17.0971458463586,20.5557114245438,-7.99685012662038));
#96314=CARTESIAN_POINT('Ctrl Pts',(17.1467942811044,20.6139667435398,-8.0011697055739));
#96315=CARTESIAN_POINT('Ctrl Pts',(17.2060220540859,20.6762858438946,-8.00626507637166));
#96316=CARTESIAN_POINT('Ctrl Pts',(17.2126111821523,20.6831261035805,-8.00683120617705));
#96317=CARTESIAN_POINT('Ctrl Pts',(17.2224462457332,20.6931994581455,-8.00767556563659));
#96318=CARTESIAN_POINT('Ctrl Pts',(17.2256571128251,20.6964668355668,-8.00795112243373));
#96319=CARTESIAN_POINT('Ctrl Pts',(17.2313903530047,20.7022632252796,-8.00844302466834));
#96320=CARTESIAN_POINT('Ctrl Pts',(17.2339085462928,20.7047963009055,-8.00865904106725));
#96321=CARTESIAN_POINT('Ctrl Pts',(17.2393381939048,20.7102304618452,-8.00912473813137));
#96322=CARTESIAN_POINT('Ctrl Pts',(17.24225164675,20.713129402627,-8.0093745743581));
#96323=CARTESIAN_POINT('Ctrl Pts',(17.2503213510491,20.7211122806969,-8.0100663901133));
#96324=CARTESIAN_POINT('Ctrl Pts',(17.255495216696,20.7261782191946,-8.01050974096148));
#96325=CARTESIAN_POINT('Ctrl Pts',(17.2840548479455,20.7538565302249,-8.01295538347109));
#96326=CARTESIAN_POINT('Ctrl Pts',(17.3079320812791,20.7759527913074,-8.01499400171965));
#96327=CARTESIAN_POINT('Ctrl Pts',(17.4542419784494,20.9052203437802,-8.02739987358347));
#96328=CARTESIAN_POINT('Ctrl Pts',(17.5881861916158,20.9985328843815,-8.03835713692242));
#96329=CARTESIAN_POINT('Ctrl Pts',(17.8343783743141,21.1308997070506,-8.05661522148226));
#96330=CARTESIAN_POINT('Ctrl Pts',(17.9416765787113,21.1776126605987,-8.06405606215507));
#96331=CARTESIAN_POINT('Ctrl Pts',(18.0658261019792,21.2198396719132,-8.07206311997383));
#96332=CARTESIAN_POINT('Ctrl Pts',(18.0794008219358,21.2243040300073,-8.07293109613394));
#96333=CARTESIAN_POINT('Ctrl Pts',(18.1010776391975,21.2311905266587,-8.07430540489296));
#96334=CARTESIAN_POINT('Ctrl Pts',(18.1091506606512,21.2337020999544,-8.07481466556056));
#96335=CARTESIAN_POINT('Ctrl Pts',(18.1234152327211,21.2380463564476,-8.07571004379625));
#96336=CARTESIAN_POINT('Ctrl Pts',(18.1296004872502,21.2398991891272,-8.07609681749158));
#96337=CARTESIAN_POINT('Ctrl Pts',(18.1424111099261,21.2436729122879,-8.07689488630773));
#96338=CARTESIAN_POINT('Ctrl Pts',(18.1490375911505,21.2455897781057,-8.07730604604789));
#96339=CARTESIAN_POINT('Ctrl Pts',(18.166070899332,21.25042696941,-8.07835875581398));
#96340=CARTESIAN_POINT('Ctrl Pts',(18.1764910177686,21.2533000681174,-8.07899876453877));
#96341=CARTESIAN_POINT('Ctrl Pts',(18.2200727323989,21.2649582772887,-8.08165942876993));
#96342=CARTESIAN_POINT('Ctrl Pts',(18.2534244858284,21.2730167829108,-8.0836565555659));
#96343=CARTESIAN_POINT('Ctrl Pts',(18.3408211698685,21.2918978747048,-8.08880062896024));
#96344=CARTESIAN_POINT('Ctrl Pts',(18.395119756103,21.3014273206944,-8.09190818665326));
#96345=CARTESIAN_POINT('Ctrl Pts',(18.558087554699,21.3235104592055,-8.10105259497788));
#96346=CARTESIAN_POINT('Ctrl Pts',(18.6674213665384,21.3297764860522,-8.10694071621996));
#96347=CARTESIAN_POINT('Ctrl Pts',(18.8224704760556,21.3266448750069,-8.11538396096906));
#96348=CARTESIAN_POINT('Ctrl Pts',(18.868148293439,21.3242402277935,-8.11788440221592));
#96349=CARTESIAN_POINT('Ctrl Pts',(18.9364182366071,21.3184238350479,-8.121683728107));
#96350=CARTESIAN_POINT('Ctrl Pts',(18.9590922383782,21.3161227506819,-8.12295594650712));
#96351=CARTESIAN_POINT('Ctrl Pts',(18.9827476317918,21.3133355293284,-8.12429799866372));
#96352=CARTESIAN_POINT('Ctrl Pts',(18.9837710919019,21.3132141812487,-8.12435609206462));
#96353=CARTESIAN_POINT('Ctrl Pts',(19.002979573237,21.3109224734936,-8.12544694983261));
#96354=CARTESIAN_POINT('Ctrl Pts',(19.0211352936121,21.3085170305476,-8.12648727956017));
#96355=CARTESIAN_POINT('Ctrl Pts',(19.0724306378924,21.3010424776495,-8.12945840902469));
#96356=CARTESIAN_POINT('Ctrl Pts',(19.1054826762905,21.2954215488278,-8.13141066199488));
#96357=CARTESIAN_POINT('Ctrl Pts',(19.1451886509711,21.2876947135554,-8.13381674319363));
#96358=CARTESIAN_POINT('Ctrl Pts',(19.1519854655372,21.2863373671765,-8.13423077766921));
#96359=CARTESIAN_POINT('Ctrl Pts',(19.1631327442401,21.2840542373189,-8.13491356382834));
#96360=CARTESIAN_POINT('Ctrl Pts',(19.1674872336785,21.2831480643169,-8.13518122117521));
#96361=CARTESIAN_POINT('Ctrl Pts',(19.1753236438988,21.2814915185107,-8.13566464617708));
#96362=CARTESIAN_POINT('Ctrl Pts',(19.1788065507276,21.2807460759703,-8.13588012973324));
#96363=CARTESIAN_POINT('Ctrl Pts',(19.186400010301,21.279100804254,-8.13635130159189));
#96364=CARTESIAN_POINT('Ctrl Pts',(19.1905097155735,21.2781975195304,-8.13660718127647));
#96365=CARTESIAN_POINT('Ctrl Pts',(19.2021221970862,21.2756088591033,-8.13733261939392));
#96366=CARTESIAN_POINT('Ctrl Pts',(19.2096184317918,21.2738948678181,-8.13780377169432));
#96367=CARTESIAN_POINT('Ctrl Pts',(19.2560133768138,21.2630204827113,-8.140736802999));
#96368=CARTESIAN_POINT('Ctrl Pts',(19.2946528830285,21.2528016295424,-8.14325373050464));
#96369=CARTESIAN_POINT('Ctrl Pts',(19.4980638283956,21.1927973433519,-8.1568181688231));
#96370=CARTESIAN_POINT('Ctrl Pts',(19.6565953930106,21.12414827831,-8.16843474910766));
#96371=CARTESIAN_POINT('Ctrl Pts',(19.8911270319894,20.986584227413,-8.18607030865468));
#96372=CARTESIAN_POINT('Ctrl Pts',(19.9735159336012,20.9300833420083,-8.19238237733184));
#96373=CARTESIAN_POINT('Ctrl Pts',(20.0625529989311,20.8592812133051,-8.19932540923305));
#96374=CARTESIAN_POINT('Ctrl Pts',(20.0733975307582,20.8504811064398,-8.20017343930853));
#96375=CARTESIAN_POINT('Ctrl Pts',(20.0905936595884,20.8362423005961,-8.20152220885994));
#96376=CARTESIAN_POINT('Ctrl Pts',(20.0970013530965,20.830872281222,-8.20202570948833));
#96377=CARTESIAN_POINT('Ctrl Pts',(20.1082896414763,20.8212976357773,-8.20291440908608));
#96378=CARTESIAN_POINT('Ctrl Pts',(20.113183140604,20.8171084523018,-8.20330023336711));
#96379=CARTESIAN_POINT('Ctrl Pts',(20.1233072365092,20.8083611164578,-8.20409968921891));
#96380=CARTESIAN_POINT('Ctrl Pts',(20.128534706106,20.8037994503438,-8.20451316885232));
#96381=CARTESIAN_POINT('Ctrl Pts',(20.1419842492729,20.791945958442,-8.20557884831614));
#96382=CARTESIAN_POINT('Ctrl Pts',(20.1501722045024,20.7846156022991,-8.20622943165243));
#96383=CARTESIAN_POINT('Ctrl Pts',(20.1848730068321,20.753059118047,-8.20899488465013));
#96384=CARTESIAN_POINT('Ctrl Pts',(20.210825083705,20.728223352771,-8.2110837944121));
#96385=CARTESIAN_POINT('Ctrl Pts',(20.2775057749932,20.6610779729768,-8.21652053183953));
#96386=CARTESIAN_POINT('Ctrl Pts',(20.3171285775791,20.6177127884411,-8.2198228258352));
#96387=CARTESIAN_POINT('Ctrl Pts',(20.4628437274544,20.444267609799,-8.23238322920137));
#96388=CARTESIAN_POINT('Ctrl Pts',(20.5551182790621,20.3034150048165,-8.24121620710234));
#96389=CARTESIAN_POINT('Ctrl Pts',(20.6314960346413,20.1497291724357,-8.25085098543962));
#96390=CARTESIAN_POINT('Ctrl Pts',(20.6331907606959,20.1462957365846,-8.25106625556775));
#96391=CARTESIAN_POINT('Ctrl Pts',(20.6577113722162,20.0962766791371,-8.25420295792358));
#96392=CARTESIAN_POINT('Ctrl Pts',(20.678824703109,20.0488759881436,-8.25718286206112));
#96393=CARTESIAN_POINT('Ctrl Pts',(20.7014034567775,19.9927209021678,-8.26077501603406));
#96394=CARTESIAN_POINT('Ctrl Pts',(20.7045833399969,19.984669971603,-8.26129148001002));
#96395=CARTESIAN_POINT('Ctrl Pts',(20.7093300393406,19.9724329986888,-8.26207900987483));
#96396=CARTESIAN_POINT('Ctrl Pts',(20.7109331643739,19.9682610108606,-8.26234794909308));
#96397=CARTESIAN_POINT('Ctrl Pts',(20.7137905577849,19.9607539883235,-8.26283272581797));
#96398=CARTESIAN_POINT('Ctrl Pts',(20.7150496273832,19.9574208392315,-8.26304827190273));
#96399=CARTESIAN_POINT('Ctrl Pts',(20.7177712210673,19.950160539718,-8.26351844693558));
#96400=CARTESIAN_POINT('Ctrl Pts',(20.7192304823261,19.9462322710219,-8.26377326102612));
#96401=CARTESIAN_POINT('Ctrl Pts',(20.7233068825824,19.9351581593428,-8.26449273281755));
#96402=CARTESIAN_POINT('Ctrl Pts',(20.7258971365562,19.9280025844964,-8.26495894379259));
#96403=CARTESIAN_POINT('Ctrl Pts',(20.7413585026825,19.8845601303327,-8.26779669235938));
#96404=CARTESIAN_POINT('Ctrl Pts',(20.7532754284984,19.847944048314,-8.27021930295199));
#96405=CARTESIAN_POINT('Ctrl Pts',(20.7896151056037,19.7249888869659,-8.2784098183297));
#96406=CARTESIAN_POINT('Ctrl Pts',(20.8095471149129,19.637427285596,-8.28432867735865));
#96407=CARTESIAN_POINT('Ctrl Pts',(20.8512543218205,19.3794525057696,-8.30159711793062));
#96408=CARTESIAN_POINT('Ctrl Pts',(20.8579468921458,19.2072970879756,-8.31284884369033));
#96409=CARTESIAN_POINT('Ctrl Pts',(20.8418510982953,19.0130266556424,-8.32485059558149));
#96410=CARTESIAN_POINT('Ctrl Pts',(20.8395493863457,18.9898856698573,-8.32627034371171));
#96411=CARTESIAN_POINT('Ctrl Pts',(20.8357605984607,18.9572612732565,-8.32825867100352));
#96412=CARTESIAN_POINT('Ctrl Pts',(20.8345896727262,18.9477434972117,-8.32883714757774));
#96413=CARTESIAN_POINT('Ctrl Pts',(20.8325842947206,18.9323090342857,-8.32977272625912));
#96414=CARTESIAN_POINT('Ctrl Pts',(20.8317894031988,18.9263874258171,-8.33013107217587));
#96415=CARTESIAN_POINT('Ctrl Pts',(20.8300749643775,18.9140130889018,-8.33087868039416));
#96416=CARTESIAN_POINT('Ctrl Pts',(20.8291506631589,18.9075610740465,-8.33126778821291));
#96417=CARTESIAN_POINT('Ctrl Pts',(20.8268846346344,18.8922473793663,-8.33218971753388));
#96418=CARTESIAN_POINT('Ctrl Pts',(20.8255163934888,18.883389703184,-8.33272169411313));
#96419=CARTESIAN_POINT('Ctrl Pts',(20.8207363892071,18.8536962049064,-8.33450092963488));
#96420=CARTESIAN_POINT('Ctrl Pts',(20.8170691270874,18.8329023680257,-8.33574008851171));
#96421=CARTESIAN_POINT('Ctrl Pts',(20.7955578853588,18.7207658163982,-8.34239075009146));
#96422=CARTESIAN_POINT('Ctrl Pts',(20.7720154745158,18.6306153875568,-8.34761651828512));
#96423=CARTESIAN_POINT('Ctrl Pts',(20.6936297918942,18.3951642806919,-8.36128220548598));
#96424=CARTESIAN_POINT('Ctrl Pts',(20.6286327564428,18.2538704220254,-8.3694817678823));
#96425=CARTESIAN_POINT('Ctrl Pts',(20.5213551863295,18.075266506892,-8.38119932045691));
#96426=CARTESIAN_POINT('Ctrl Pts',(20.4922016398175,18.0306377222315,-8.38425744364819));
#96427=CARTESIAN_POINT('Ctrl Pts',(20.4563594469984,17.9800479644633,-8.38793672734164));
#96428=CARTESIAN_POINT('Ctrl Pts',(20.4512766133898,17.9729668802289,-8.3884567441382));
#96429=CARTESIAN_POINT('Ctrl Pts',(20.4435140126833,17.9622922949229,-8.38924863379105));
#96430=CARTESIAN_POINT('Ctrl Pts',(20.4408662513414,17.9586754847638,-8.3895183445052));
#96431=CARTESIAN_POINT('Ctrl Pts',(20.4360927148667,17.9521981523849,-8.39000393956645));
#96432=CARTESIAN_POINT('Ctrl Pts',(20.4339711870085,17.9493345670877,-8.3902195280915));
#96433=CARTESIAN_POINT('Ctrl Pts',(20.4293453335256,17.9431235562909,-8.39068912492562));
#96434=CARTESIAN_POINT('Ctrl Pts',(20.4268383533856,17.9397782313739,-8.39094331470733));
#96435=CARTESIAN_POINT('Ctrl Pts',(20.4197678472627,17.9304013231137,-8.39165929895434));
#96436=CARTESIAN_POINT('Ctrl Pts',(20.4151819356171,17.9243868096831,-8.39212262318725));
#96437=CARTESIAN_POINT('Ctrl Pts',(20.3875576544783,17.8885568771406,-8.39490660566813));
#96438=CARTESIAN_POINT('Ctrl Pts',(20.3637603617581,17.8593382495859,-8.3972761613492));
#96439=CARTESIAN_POINT('Ctrl Pts',(20.2828441327697,17.765233076241,-8.40519900828723));
#96440=CARTESIAN_POINT('Ctrl Pts',(20.222532794194,17.7032107692611,-8.41089346404166));
#96441=CARTESIAN_POINT('Ctrl Pts',(20.0282225120172,17.5264390366334,-8.42824879052193));
#96442=CARTESIAN_POINT('Ctrl Pts',(19.8835097537651,17.4245485897652,-8.43982447440901));
#96443=CARTESIAN_POINT('Ctrl Pts',(19.7075711575063,17.331006923692,-8.45208853724492));
#96444=CARTESIAN_POINT('Ctrl Pts',(19.687151087674,17.3205720498639,-8.45348825398657));
#96445=CARTESIAN_POINT('Ctrl Pts',(19.6580039328834,17.3062699225899,-8.45545360106586));
#96446=CARTESIAN_POINT('Ctrl Pts',(19.6494146069852,17.3021270241979,-8.45602882258404));
#96447=CARTESIAN_POINT('Ctrl Pts',(19.6354074198043,17.2954872111137,-8.45696056837813));
#96448=CARTESIAN_POINT('Ctrl Pts',(19.6300065530493,17.2929549434672,-8.45731831645653));
#96449=CARTESIAN_POINT('Ctrl Pts',(19.6186744877923,17.2877000647936,-8.45806580946481));
#96450=CARTESIAN_POINT('Ctrl Pts',(19.6127412494342,17.2849819813592,-8.45845539494049));
#96451=CARTESIAN_POINT('Ctrl Pts',(19.5985882225104,17.2785773343802,-8.45938050958642));
#96452=CARTESIAN_POINT('Ctrl Pts',(19.5903572422829,17.274915696434,-8.45991517790893));
#96453=CARTESIAN_POINT('Ctrl Pts',(19.5625100943552,17.2627399310947,-8.46171300575328));
#96454=CARTESIAN_POINT('Ctrl Pts',(19.542787970593,17.2544703323282,-8.46296782850978));
#96455=CARTESIAN_POINT('Ctrl Pts',(19.4344865306406,17.2109764472891,-8.46976380966929));
#96456=CARTESIAN_POINT('Ctrl Pts',(19.3437260174913,17.1814648699934,-8.47510959358759));
#96457=CARTESIAN_POINT('Ctrl Pts',(19.0858065025412,17.1164738235139,-8.48974106747186));
#96458=CARTESIAN_POINT('Ctrl Pts',(18.9159230842882,17.0949424352635,-8.49871735792444));
#96459=CARTESIAN_POINT('Ctrl Pts',(18.7086783881462,17.0938343522178,-8.51055653629938));
#96460=CARTESIAN_POINT('Ctrl Pts',(18.672041428243,17.094589752273,-8.51268514326574));
#96461=CARTESIAN_POINT('Ctrl Pts',(18.6283201407103,17.0966273643405,-8.5152873411395));
#96462=CARTESIAN_POINT('Ctrl Pts',(18.6211970346115,17.0969954203394,-8.51571326305379));
#96463=CARTESIAN_POINT('Ctrl Pts',(18.6095737373756,17.0976549166907,-8.51641168402998));
#96464=CARTESIAN_POINT('Ctrl Pts',(18.6050723113554,17.0979247561399,-8.51668300189247));
#96465=CARTESIAN_POINT('Ctrl Pts',(18.5970131019333,17.0984337158775,-8.51717031272833));
#96466=CARTESIAN_POINT('Ctrl Pts',(18.5934550311703,17.0986674441479,-8.51738600072837));
#96467=CARTESIAN_POINT('Ctrl Pts',(18.5857471058617,17.0991933361385,-8.51785444316563));
#96468=CARTESIAN_POINT('Ctrl Pts',(18.5815975733909,17.0994887388824,-8.51810737162843));
#96469=CARTESIAN_POINT('Ctrl Pts',(18.5699997810276,17.1003487441403,-8.5188163272104));
#96470=CARTESIAN_POINT('Ctrl Pts',(18.5625536846635,17.1009405333451,-8.51927383721742));
#96471=CARTESIAN_POINT('Ctrl Pts',(18.5191536764231,17.1046210490033,-8.52195350479844));
#96472=CARTESIAN_POINT('Ctrl Pts',(18.4832826039097,17.1085890849786,-8.52422047812991));
#96473=CARTESIAN_POINT('Ctrl Pts',(18.3679222706884,17.1243442570112,-8.53164286914908));
#96474=CARTESIAN_POINT('Ctrl Pts',(18.2890001702411,17.139739870969,-8.53692186007904));
#96475=CARTESIAN_POINT('Ctrl Pts',(18.0316459477705,17.2053323900169,-8.5544565935549));
#96476=CARTESIAN_POINT('Ctrl Pts',(17.8588819769178,17.2744567631978,-8.56666089245527));
#96477=CARTESIAN_POINT('Ctrl Pts',(17.6780092373775,17.376044322465,-8.57941891882172));
#96478=CARTESIAN_POINT('Ctrl Pts',(17.6588830642299,17.387184641459,-8.58076925482921));
#96479=CARTESIAN_POINT('Ctrl Pts',(17.6320449020001,17.4033858566895,-8.58266649424393));
#96480=CARTESIAN_POINT('Ctrl Pts',(17.6241863729939,17.4082000536342,-8.58322233113494));
#96481=CARTESIAN_POINT('Ctrl Pts',(17.6108614664833,17.4164831450663,-8.58416540336677));
#96482=CARTESIAN_POINT('Ctrl Pts',(17.6053791590805,17.4199260464738,-8.58455358817342));
#96483=CARTESIAN_POINT('Ctrl Pts',(17.5944481450155,17.4268608659521,-8.58532796368129));
#96484=CARTESIAN_POINT('Ctrl Pts',(17.5889994863794,17.4303527286176,-8.58571415084382));
#96485=CARTESIAN_POINT('Ctrl Pts',(17.5780647883964,17.4374313528938,-8.58648960508637));
#96486=CARTESIAN_POINT('Ctrl Pts',(17.572579223143,17.4410187176184,-8.58687884406315));
#96487=CARTESIAN_POINT('Ctrl Pts',(17.5527646003415,17.4541085561743,-8.58828571269778));
#96488=CARTESIAN_POINT('Ctrl Pts',(17.5385345249328,17.4637601942952,-8.58929774595583));
#96489=CARTESIAN_POINT('Ctrl Pts',(17.4031522189394,17.5580124148171,-8.59894690493272));
#96490=CARTESIAN_POINT('Ctrl Pts',(17.2910488158158,17.6549076223824,-8.60705901703929));
#96491=CARTESIAN_POINT('Ctrl Pts',(17.0877647716834,17.8716328738512,-8.62320800980143));
#96492=CARTESIAN_POINT('Ctrl Pts',(16.9974183756671,17.9910548564931,-8.63121057716827));
#96493=CARTESIAN_POINT('Ctrl Pts',(16.9122949762965,18.1324237944112,-8.6408855694134));
#96494=CARTESIAN_POINT('Ctrl Pts',(16.904341119639,18.1459722193693,-8.6418149038339));
#96495=CARTESIAN_POINT('Ctrl Pts',(16.8936618097339,18.1646358622268,-8.64309973931608));
#96496=CARTESIAN_POINT('Ctrl Pts',(16.8908052566807,18.1696759871327,-8.64344716685032));
#96497=CARTESIAN_POINT('Ctrl Pts',(16.8862994306781,18.1777027310987,-8.64400129639221));
#96498=CARTESIAN_POINT('Ctrl Pts',(16.8846366033134,18.1806817644988,-8.64420713536483));
#96499=CARTESIAN_POINT('Ctrl Pts',(16.8812176602314,18.1868419043327,-8.64463317458206));
#96500=CARTESIAN_POINT('Ctrl Pts',(16.8794625363721,18.1900235072734,-8.64485343834559));
#96501=CARTESIAN_POINT('Ctrl Pts',(16.8753006132713,18.1976141787908,-8.64537944795096));
#96502=CARTESIAN_POINT('Ctrl Pts',(16.8729013065442,18.2020273121253,-8.64568566673566));
#96503=CARTESIAN_POINT('Ctrl Pts',(16.8648653629559,18.2169343069357,-8.64672128030589));
#96504=CARTESIAN_POINT('Ctrl Pts',(16.8593017156538,18.2274669699382,-8.6474550757251));
#96505=CARTESIAN_POINT('Ctrl Pts',(16.8124639527543,18.3179779859893,-8.65377488464604));
#96506=CARTESIAN_POINT('Ctrl Pts',(16.7762596204173,18.400428355294,-8.65962160080874));
#96507=CARTESIAN_POINT('Ctrl Pts',(16.745419494333,18.4848894213129,-8.66553665550751));
#96508=CARTESIAN_POINT('',(16.6172480928634,19.2105366953923,-7.68905625083793));
#96509=CARTESIAN_POINT('Ctrl Pts',(16.7454194503191,18.4848895418526,-8.44448864899009));
#96510=CARTESIAN_POINT('Ctrl Pts',(16.7701773779263,18.4170856247798,-8.44016252686615));
#96511=CARTESIAN_POINT('Ctrl Pts',(16.7983989656721,18.3505720253294,-8.43583640474221));
#96512=CARTESIAN_POINT('Ctrl Pts',(16.8299125180811,18.2857217385025,-8.43151028261827));
#96513=CARTESIAN_POINT('Ctrl Pts',(16.8614397445838,18.2208433123886,-8.42718228334008));
#96514=CARTESIAN_POINT('Ctrl Pts',(16.8962615406801,18.1576300696997,-8.42285428406188));
#96515=CARTESIAN_POINT('Ctrl Pts',(16.934160677018,18.0964294946269,-8.41852628478368));
#96516=CARTESIAN_POINT('Ctrl Pts',(16.9721294358797,18.0351164911742,-8.41419033476406));
#96517=CARTESIAN_POINT('Ctrl Pts',(17.0131865452822,17.9758239484975,-8.40985438474445));
#96518=CARTESIAN_POINT('Ctrl Pts',(17.0570722997309,17.9188690128048,-8.40551843472483));
#96519=CARTESIAN_POINT('Ctrl Pts',(17.097271661252,17.8666982781533,-8.40154670347478));
#96520=CARTESIAN_POINT('Ctrl Pts',(17.1398437335012,17.8164887482056,-8.39757497222472));
#96521=CARTESIAN_POINT('Ctrl Pts',(17.1845622179524,17.7684565657966,-8.39360324097467));
#96522=CARTESIAN_POINT('Ctrl Pts',(17.2339699045481,17.715387705255,-8.38921503204377));
#96523=CARTESIAN_POINT('Ctrl Pts',(17.2862036327226,17.6647565409339,-8.38482682311287));
#96524=CARTESIAN_POINT('Ctrl Pts',(17.3409933109755,17.6168791249303,-8.38043861418197));
#96525=CARTESIAN_POINT('Ctrl Pts',(17.3957016722614,17.5690727669504,-8.37605691808071));
#96526=CARTESIAN_POINT('Ctrl Pts',(17.4529580928698,17.5240123587828,-8.37167522197945));
#96527=CARTESIAN_POINT('Ctrl Pts',(17.5124544762691,17.4819784462151,-8.36729352587818));
#96528=CARTESIAN_POINT('Ctrl Pts',(17.5718809466829,17.4399939268397,-8.36291697861854));
#96529=CARTESIAN_POINT('Ctrl Pts',(17.6335417591175,17.4010291152648,-8.35854043135889));
#96530=CARTESIAN_POINT('Ctrl Pts',(17.6970957742214,17.3653243441595,-8.35416388409925));
#96531=CARTESIAN_POINT('Ctrl Pts',(17.7606094842925,17.3296422165011,-8.34979011238228));
#96532=CARTESIAN_POINT('Ctrl Pts',(17.826013595285,17.29721626287,-8.3454163406653));
#96533=CARTESIAN_POINT('Ctrl Pts',(17.8929392167475,17.2682427431934,-8.34104256894832));
#96534=CARTESIAN_POINT('Ctrl Pts',(17.9598444725186,17.2392780402562,-8.33667012818477));
#96535=CARTESIAN_POINT('Ctrl Pts',(18.0282698771516,17.2137638770621,-8.33229768742122));
#96536=CARTESIAN_POINT('Ctrl Pts',(18.0978247669405,17.1918491703586,-8.32792524665767));
#96537=CARTESIAN_POINT('Ctrl Pts',(18.1673814352556,17.1699339032935,-8.32355269409032));
#96538=CARTESIAN_POINT('Ctrl Pts',(18.2380671853845,17.1516184185037,-8.31918014152297));
#96539=CARTESIAN_POINT('Ctrl Pts',(18.3094759435897,17.1370018501626,-8.31480758895562));
#96540=CARTESIAN_POINT('Ctrl Pts',(18.3809588124976,17.1223701121955,-8.31043049838829));
#96541=CARTESIAN_POINT('Ctrl Pts',(18.4531657140458,17.1114450521883,-8.30605340782097));
#96542=CARTESIAN_POINT('Ctrl Pts',(18.5256809453885,17.1042745381788,-8.30167631725364));
#96543=CARTESIAN_POINT('Ctrl Pts',(18.5982357799905,17.0971001080854,-8.2972968361947));
#96544=CARTESIAN_POINT('Ctrl Pts',(18.6710987974679,17.0936843291133,-8.29291735513576));
#96545=CARTESIAN_POINT('Ctrl Pts',(18.7438524696358,17.0940229267084,-8.28853787407681));
#96546=CARTESIAN_POINT('Ctrl Pts',(18.8167350971993,17.0943621244655,-8.28415063041709));
#96547=CARTESIAN_POINT('Ctrl Pts',(18.8895075103792,17.0984689605669,-8.27976338675737));
#96548=CARTESIAN_POINT('Ctrl Pts',(18.9617560690979,17.1062871518924,-8.27537614309765));
#96549=CARTESIAN_POINT('Ctrl Pts',(19.0108781271719,17.1116027686346,-8.27239324016285));
#96550=CARTESIAN_POINT('Ctrl Pts',(19.0597581560643,17.1186329436866,-8.26941033722804));
#96551=CARTESIAN_POINT('Ctrl Pts',(19.1082694567067,17.1273466282089,-8.26642743429323));
#96552=CARTESIAN_POINT('Ctrl Pts',(19.1796354137562,17.1401655060193,-8.26203922536233));
#96553=CARTESIAN_POINT('Ctrl Pts',(19.2504813367647,17.1566801162964,-8.25765101643143));
#96554=CARTESIAN_POINT('Ctrl Pts',(19.3203952805281,17.1768344278367,-8.25326280750054));
#96555=CARTESIAN_POINT('Ctrl Pts',(19.3902054604072,17.1969588270371,-8.24888111139927));
#96556=CARTESIAN_POINT('Ctrl Pts',(19.4590859472334,17.2207120714409,-8.244499415298));
#96557=CARTESIAN_POINT('Ctrl Pts',(19.5266340795879,17.2479869547362,-8.24011771919673));
#96558=CARTESIAN_POINT('Ctrl Pts',(19.5941028375111,17.2752297878729,-8.23574117193709));
#96559=CARTESIAN_POINT('Ctrl Pts',(19.6602419060114,17.3059858596158,-8.23136462467746));
#96560=CARTESIAN_POINT('Ctrl Pts',(19.7246645510869,17.3400984132724,-8.22698807741783));
#96561=CARTESIAN_POINT('Ctrl Pts',(19.7890463402572,17.3741893332433,-8.22261430570085));
#96562=CARTESIAN_POINT('Ctrl Pts',(19.8517134405357,17.4116322864694,-8.21824053398388));
#96563=CARTESIAN_POINT('Ctrl Pts',(19.9123011549776,17.4522233262354,-8.2138667622669));
#96564=CARTESIAN_POINT('Ctrl Pts',(19.9728704323745,17.4928020140117,-8.20949432150335));
#96565=CARTESIAN_POINT('Ctrl Pts',(20.0313611796543,17.5365266181305,-8.2051218807398));
#96566=CARTESIAN_POINT('Ctrl Pts',(20.0874367225443,17.5831492580496,-8.20074943997625));
#96567=CARTESIAN_POINT('Ctrl Pts',(20.1435136992921,17.6297730901147,-8.19637688740891));
#96568=CARTESIAN_POINT('Ctrl Pts',(20.1971749793953,17.6792947951744,-8.19200433484157));
#96569=CARTESIAN_POINT('Ctrl Pts',(20.2481174066903,17.7314265889259,-8.18763178227423));
#96570=CARTESIAN_POINT('Ctrl Pts',(20.2991127039579,17.7836124870194,-8.18325469170691));
#96571=CARTESIAN_POINT('Ctrl Pts',(20.3473831767916,17.8384135364598,-8.17887760113958));
#96572=CARTESIAN_POINT('Ctrl Pts',(20.3926635636808,17.895506107001,-8.17450051057226));
#96573=CARTESIAN_POINT('Ctrl Pts',(20.43796867987,17.952629857914,-8.17012102951332));
#96574=CARTESIAN_POINT('Ctrl Pts',(20.4802801788309,18.0120472284178,-8.16574154845437));
#96575=CARTESIAN_POINT('Ctrl Pts',(20.5193756546996,18.073404829649,-8.16136206739543));
#96576=CARTESIAN_POINT('Ctrl Pts',(20.5585404270369,18.1348711868165,-8.15697482373571));
#96577=CARTESIAN_POINT('Ctrl Pts',(20.5944775548128,18.1982842223061,-8.15258758007599));
#96578=CARTESIAN_POINT('Ctrl Pts',(20.6270104676959,18.263265665287,-8.14820033641627));
#96579=CARTESIAN_POINT('Ctrl Pts',(20.6491297135924,18.3074467849172,-8.14521743348144));
#96580=CARTESIAN_POINT('Ctrl Pts',(20.6696762814795,18.3523524542015,-8.14223453054662));
#96581=CARTESIAN_POINT('Ctrl Pts',(20.688607698715,18.3978593331261,-8.13925162761179));
#96582=CARTESIAN_POINT('Ctrl Pts',(20.7164580900963,18.4648054245267,-8.1348634186809));
#96583=CARTESIAN_POINT('Ctrl Pts',(20.7409194707723,18.5333146794851,-8.13047520975));
#96584=CARTESIAN_POINT('Ctrl Pts',(20.7618159759921,18.6030103886487,-8.1260870008191));
#96585=CARTESIAN_POINT('Ctrl Pts',(20.7826814673335,18.6726026578242,-8.12170530471784));
#96586=CARTESIAN_POINT('Ctrl Pts',(20.7999924489196,18.7433774273515,-8.11732360861657));
#96587=CARTESIAN_POINT('Ctrl Pts',(20.813621111304,18.8149380939565,-8.1129419125153));
#96588=CARTESIAN_POINT('Ctrl Pts',(20.8272337589254,18.8864146710833,-8.10856536525567));
#96589=CARTESIAN_POINT('Ctrl Pts',(20.8371725931962,18.9586748392569,-8.10418881799603));
#96590=CARTESIAN_POINT('Ctrl Pts',(20.8433600899068,19.0313085669594,-8.09981227073639));
#96591=CARTESIAN_POINT('Ctrl Pts',(20.849543662597,19.1038962314074,-8.09543849901942));
#96592=CARTESIAN_POINT('Ctrl Pts',(20.8519805772149,19.1768565058775,-8.09106472730244));
#96593=CARTESIAN_POINT('Ctrl Pts',(20.8506449171335,19.2497723454649,-8.08669095558546));
#96594=CARTESIAN_POINT('Ctrl Pts',(20.8493096634979,19.3226659965175,-8.08231851482191));
#96595=CARTESIAN_POINT('Ctrl Pts',(20.8442041231404,19.3955147575252,-8.07794607405835));
#96596=CARTESIAN_POINT('Ctrl Pts',(20.8353544889708,19.4679013656687,-8.07357363329479));
#96597=CARTESIAN_POINT('Ctrl Pts',(20.826504628515,19.5402898247457,-8.06920108072744));
#96598=CARTESIAN_POINT('Ctrl Pts',(20.8139105446927,19.6122156289264,-8.06482852816009));
#96599=CARTESIAN_POINT('Ctrl Pts',(20.797650125878,19.6832680996678,-8.06045597559274));
#96600=CARTESIAN_POINT('Ctrl Pts',(20.7813728313873,19.7543943113433,-8.05607888502542));
#96601=CARTESIAN_POINT('Ctrl Pts',(20.761421712685,19.8246449087065,-8.05170179445809));
#96602=CARTESIAN_POINT('Ctrl Pts',(20.7379253105676,19.8936216738915,-8.04732470389076));
#96603=CARTESIAN_POINT('Ctrl Pts',(20.7144160761931,19.962636109848,-8.04294522283182));
#96604=CARTESIAN_POINT('Ctrl Pts',(20.6873578824886,20.0303748802483,-8.03856574177289));
#96605=CARTESIAN_POINT('Ctrl Pts',(20.6569274894875,20.0964596942681,-8.03418626071395));
#96606=CARTESIAN_POINT('Ctrl Pts',(20.626443158819,20.1626616431772,-8.02979901705423));
#96607=CARTESIAN_POINT('Ctrl Pts',(20.5925749169663,20.2272033538502,-8.02541177339451));
#96608=CARTESIAN_POINT('Ctrl Pts',(20.5555452556637,20.2897316077547,-8.02102452973479));
#96609=CARTESIAN_POINT('Ctrl Pts',(20.5303686541477,20.3322447952014,-8.01804162679998));
#96610=CARTESIAN_POINT('Ctrl Pts',(20.5037315602568,20.3738277943096,-8.01505872386517));
#96611=CARTESIAN_POINT('Ctrl Pts',(20.475714693788,20.4143781306983,-8.01207582093037));
#96612=CARTESIAN_POINT('Ctrl Pts',(20.434498513999,20.4740325519721,-8.00768761199947));
#96613=CARTESIAN_POINT('Ctrl Pts',(20.3901335538168,20.5316834623514,-8.00329940306858));
#96614=CARTESIAN_POINT('Ctrl Pts',(20.3428413739373,20.5869790817842,-7.99891119413768));
#96615=CARTESIAN_POINT('Ctrl Pts',(20.2956193834939,20.6421926333496,-7.99452949803642));
#96616=CARTESIAN_POINT('Ctrl Pts',(20.2454791086754,20.6950574697367,-7.99014780193516));
#96617=CARTESIAN_POINT('Ctrl Pts',(20.1926848492423,20.7452514495972,-7.9857661058339));
#96618=CARTESIAN_POINT('Ctrl Pts',(20.1399526272655,20.7953864475368,-7.98138955857427));
#96619=CARTESIAN_POINT('Ctrl Pts',(20.0845729637369,20.8428564928138,-7.97701301131463));
#96620=CARTESIAN_POINT('Ctrl Pts',(20.0268486678901,20.8873744575526,-7.972636464055));
#96621=CARTESIAN_POINT('Ctrl Pts',(19.9691609799528,20.9318641896452,-7.96826269233803));
#96622=CARTESIAN_POINT('Ctrl Pts',(19.9091319910002,20.9734052619583,-7.96388892062106));
#96623=CARTESIAN_POINT('Ctrl Pts',(19.8470983416198,21.011750144213,-7.95951514890408));
#96624=CARTESIAN_POINT('Ctrl Pts',(19.7850835692872,21.0500833579913,-7.95514270814054));
#96625=CARTESIAN_POINT('Ctrl Pts',(19.721065757685,21.0852220591673,-7.95077026737699));
#96626=CARTESIAN_POINT('Ctrl Pts',(19.6554099365361,21.116962415383,-7.94639782661344));
#96627=CARTESIAN_POINT('Ctrl Pts',(19.5897524365606,21.1487035832031,-7.94202527404609));
#96628=CARTESIAN_POINT('Ctrl Pts',(19.5224572790426,21.1770460253878,-7.93765272147875));
#96629=CARTESIAN_POINT('Ctrl Pts',(19.4539119391454,21.2018329412274,-7.9332801689114));
#96630=CARTESIAN_POINT('Ctrl Pts',(19.3852954603089,21.2266455818631,-7.92890307834408));
#96631=CARTESIAN_POINT('Ctrl Pts',(19.3154266631738,21.2478951643122,-7.92452598777675));
#96632=CARTESIAN_POINT('Ctrl Pts',(19.2447099626414,21.2654742232646,-7.92014889720943));
#96633=CARTESIAN_POINT('Ctrl Pts',(19.1739546410942,21.2830628827936,-7.91576941615049));
#96634=CARTESIAN_POINT('Ctrl Pts',(19.1023509680274,21.2969769355905,-7.91138993509155));
#96635=CARTESIAN_POINT('Ctrl Pts',(19.0303127030118,21.307160247222,-7.90701045403261));
#96636=CARTESIAN_POINT('Ctrl Pts',(18.958146750655,21.317361608705,-7.90262321037289));
#96637=CARTESIAN_POINT('Ctrl Pts',(18.8855451489733,21.3238189809293,-7.89823596671317));
#96638=CARTESIAN_POINT('Ctrl Pts',(18.8129253294104,21.3265282537412,-7.89384872305345));
#96639=CARTESIAN_POINT('Ctrl Pts',(18.7635508497363,21.3283702981885,-7.89086582011861));
#96640=CARTESIAN_POINT('Ctrl Pts',(18.7141679744274,21.328480806371,-7.88788291718377));
#96641=CARTESIAN_POINT('Ctrl Pts',(18.6649065603161,21.3268721834252,-7.88490001424893));
#96642=CARTESIAN_POINT('Ctrl Pts',(18.5924370961484,21.3245057056244,-7.88051180531802));
#96643=CARTESIAN_POINT('Ctrl Pts',(18.519947892475,21.3184071393706,-7.87612359638712));
#96644=CARTESIAN_POINT('Ctrl Pts',(18.4478546672516,21.3085723702762,-7.87173538745621));
#96645=CARTESIAN_POINT('Ctrl Pts',(18.3758684403278,21.2987521976098,-7.86735369135494));
#96646=CARTESIAN_POINT('Ctrl Pts',(18.3042774991941,21.2852068946333,-7.86297199525367));
#96647=CARTESIAN_POINT('Ctrl Pts',(18.233495774192,21.2679843266171,-7.8585902991524));
#96648=CARTESIAN_POINT('Ctrl Pts',(18.1627972233498,21.2507819964889,-7.85421375189275));
#96649=CARTESIAN_POINT('Ctrl Pts',(18.0929064660596,21.2299110986508,-7.84983720463311));
#96650=CARTESIAN_POINT('Ctrl Pts',(18.0242288363209,21.2054708308746,-7.84546065737347));
#96651=CARTESIAN_POINT('Ctrl Pts',(17.9555947609369,21.181046062761,-7.8410868856565));
#96652=CARTESIAN_POINT('Ctrl Pts',(17.8881727399585,21.1530565773997,-7.83671311393953));
#96653=CARTESIAN_POINT('Ctrl Pts',(17.8223531243431,21.1216514528048,-7.83233934222256));
#96654=CARTESIAN_POINT('Ctrl Pts',(17.7565535378578,21.0902558848948,-7.82796690145901));
#96655=CARTESIAN_POINT('Ctrl Pts',(17.6923558237623,21.055446948864,-7.82359446069545));
#96656=CARTESIAN_POINT('Ctrl Pts',(17.6301289564784,21.0174212463528,-7.8192220199319));
#96657=CARTESIAN_POINT('Ctrl Pts',(17.5679004980465,20.97939457152,-7.81484946736455));
#96658=CARTESIAN_POINT('Ctrl Pts',(17.507643397047,20.9381512201345,-7.81047691479719));
#96659=CARTESIAN_POINT('Ctrl Pts',(17.4496992310191,20.8939321242388,-7.80610436222984));
#96660=CARTESIAN_POINT('Ctrl Pts',(17.3916949283502,20.8496671360977,-7.80172727166251));
#96661=CARTESIAN_POINT('Ctrl Pts',(17.3360087376072,20.8024205306333,-7.79735018109518));
#96662=CARTESIAN_POINT('Ctrl Pts',(17.2829499222247,20.7524741878437,-7.79297309052785));
#96663=CARTESIAN_POINT('Ctrl Pts',(17.2298621294539,20.7025005675026,-7.78859360946891));
#96664=CARTESIAN_POINT('Ctrl Pts',(17.1794049028384,20.6498246228583,-7.78421412840997));
#96665=CARTESIAN_POINT('Ctrl Pts',(17.1318494027612,20.5947638757271,-7.77983464735103));
#96666=CARTESIAN_POINT('Ctrl Pts',(17.0842096108792,20.5396055337911,-7.7754474036913));
#96667=CARTESIAN_POINT('Ctrl Pts',(17.0394821127479,20.4820543293405,-7.77106016003157));
#96668=CARTESIAN_POINT('Ctrl Pts',(16.9978963120791,20.4224590314111,-7.76667291637185));
#96669=CARTESIAN_POINT('Ctrl Pts',(16.9696219748229,20.3819399714089,-7.76369001343706));
#96670=CARTESIAN_POINT('Ctrl Pts',(16.9427990411458,20.3404766042676,-7.76070711050228));
#96671=CARTESIAN_POINT('Ctrl Pts',(16.9174873693318,20.2981848336979,-7.75772420756749));
#96672=CARTESIAN_POINT('Ctrl Pts',(16.8789674908494,20.2338242543132,-7.75318475796429));
#96673=CARTESIAN_POINT('Ctrl Pts',(16.8438078846742,20.1673074236144,-7.74864530836108));
#96674=CARTESIAN_POINT('Ctrl Pts',(16.812247200043,20.0990062926902,-7.74410585875788));
#96675=CARTESIAN_POINT('Ctrl Pts',(16.7803526868132,20.0299827163854,-7.73951839377993));
#96676=CARTESIAN_POINT('Ctrl Pts',(16.7521339850624,19.9591372097164,-7.73493092880198));
#96677=CARTESIAN_POINT('Ctrl Pts',(16.7277918950442,19.8868831552936,-7.73034346382403));
#96678=CARTESIAN_POINT('Ctrl Pts',(16.7037989805435,19.8156655503633,-7.72582180381421));
#96679=CARTESIAN_POINT('Ctrl Pts',(16.6835723608136,19.7430799630089,-7.72130014380438));
#96680=CARTESIAN_POINT('Ctrl Pts',(16.667257251386,19.6695448844459,-7.71677848379455));
#96681=CARTESIAN_POINT('Ctrl Pts',(16.6505859845118,19.5944045413927,-7.71215811633255));
#96682=CARTESIAN_POINT('Ctrl Pts',(16.6379992287985,19.5182731789951,-7.70753774887054));
#96683=CARTESIAN_POINT('Ctrl Pts',(16.6295984951253,19.441615060829,-7.70291738140853));
#96684=CARTESIAN_POINT('Ctrl Pts',(16.6211977614521,19.3649569426629,-7.69829701394652));
#96685=CARTESIAN_POINT('Ctrl Pts',(16.6169831628437,19.2877725479369,-7.69367664648452));
#96686=CARTESIAN_POINT('Ctrl Pts',(16.617000050606,19.2105371115439,-7.68905627902251));
#96687=CARTESIAN_POINT('Ctrl Pts',(16.6203930058439,19.2105314190313,-7.68905589348729));
#96688=CARTESIAN_POINT('Ctrl Pts',(16.6199117136336,18.9629932582392,-7.67422393560445));
#96689=CARTESIAN_POINT('Ctrl Pts',(16.6606020170419,18.7156058265681,-7.65939197772161));
#96690=CARTESIAN_POINT('Ctrl Pts',(16.743090251011,18.4840590306076,-7.64456001983877));
#96691=CARTESIAN_POINT('Origin',(18.734,19.211,0.));
#96692=CARTESIAN_POINT('',(16.7454194487812,18.4848895460645,-6.84500598950246));
#96693=CARTESIAN_POINT('',(16.7454194586292,18.4848895190942,-7.06814843723424));
#96694=CARTESIAN_POINT('',(16.7454194503191,18.4848895418526,0.));
#96695=CARTESIAN_POINT('',(16.6170002518879,19.2120327115197,-7.10922273934007));
#96696=CARTESIAN_POINT('Ctrl Pts',(16.7454194586292,18.4848895190942,-7.06814843723424));
#96697=CARTESIAN_POINT('Ctrl Pts',(16.720259549706,18.553794329895,-7.07236993224033));
#96698=CARTESIAN_POINT('Ctrl Pts',(16.6986924511745,18.6239752665951,-7.07647898186573));
#96699=CARTESIAN_POINT('Ctrl Pts',(16.6383405809316,18.864188984939,-7.09013449006123));
#96700=CARTESIAN_POINT('Ctrl Pts',(16.6169152552473,19.0377944433565,-7.0992858278884));
#96701=CARTESIAN_POINT('Ctrl Pts',(16.6170002518879,19.2120327115197,-7.10922273934007));
#96702=CARTESIAN_POINT('Ctrl Pts',(16.6170002532712,19.2120355434925,-7.10922290084922));
#96703=CARTESIAN_POINT('Ctrl Pts',(16.6170133612054,19.2388325765887,-7.11075115282299));
#96704=CARTESIAN_POINT('Ctrl Pts',(16.6175352640855,19.2656259751736,-7.11229810151296));
#96705=CARTESIAN_POINT('Ctrl Pts',(16.619122764669,19.3068815384912,-7.11471891962847));
#96706=CARTESIAN_POINT('Ctrl Pts',(16.6198286091479,19.3213553104517,-7.11557560729638));
#96707=CARTESIAN_POINT('Ctrl Pts',(16.6209600187579,19.3405110738338,-7.11672054129347));
#96708=CARTESIAN_POINT('Ctrl Pts',(16.6212526901485,19.3452009103681,-7.11700173529727));
#96709=CARTESIAN_POINT('Ctrl Pts',(16.6217938177709,19.3534311768807,-7.11749681939946));
#96710=CARTESIAN_POINT('Ctrl Pts',(16.6220355692633,19.3569720496406,-7.11771034150998));
#96711=CARTESIAN_POINT('Ctrl Pts',(16.6225281743165,19.3639296116612,-7.11813095670815));
#96712=CARTESIAN_POINT('Ctrl Pts',(16.6227784202938,19.367346340043,-7.11833801621373));
#96713=CARTESIAN_POINT('Ctrl Pts',(16.6233330675212,19.3746749694206,-7.11878324617352));
#96714=CARTESIAN_POINT('Ctrl Pts',(16.6236400496941,19.3785866195106,-7.11902155756046));
#96715=CARTESIAN_POINT('Ctrl Pts',(16.6244765277737,19.3888783464362,-7.11965028919192));
#96716=CARTESIAN_POINT('Ctrl Pts',(16.6250240887253,19.3952568566875,-7.12004170273131));
#96717=CARTESIAN_POINT('Ctrl Pts',(16.6274167975964,19.4217202404669,-7.12167257857668));
#96718=CARTESIAN_POINT('Ctrl Pts',(16.6295199353153,19.441779975436,-7.12292547305272));
#96719=CARTESIAN_POINT('Ctrl Pts',(16.6324142650628,19.4660383676236,-7.12445835148569));
#96720=CARTESIAN_POINT('Ctrl Pts',(16.632932050339,19.470269436252,-7.12472636680322));
#96721=CARTESIAN_POINT('Ctrl Pts',(16.6366907788312,19.5002329405034,-7.12662890698868));
#96722=CARTESIAN_POINT('Ctrl Pts',(16.6403914564329,19.525904456337,-7.12828250345181));
#96723=CARTESIAN_POINT('Ctrl Pts',(16.6730372178307,19.7262310244932,-7.14133933788202));
#96724=CARTESIAN_POINT('Ctrl Pts',(16.7233160802222,19.8967032727669,-7.15328953573802));
#96725=CARTESIAN_POINT('Ctrl Pts',(16.8178243006676,20.1129025733623,-7.16850117879059));
#96726=CARTESIAN_POINT('Ctrl Pts',(16.8436568825246,20.1658620055677,-7.17224015923375));
#96727=CARTESIAN_POINT('Ctrl Pts',(16.8887823512088,20.2493430978163,-7.1781470852501));
#96728=CARTESIAN_POINT('Ctrl Pts',(16.9067037348598,20.2805668138392,-7.18035976692358));
#96729=CARTESIAN_POINT('Ctrl Pts',(16.9311299514349,20.3207159778056,-7.18321120806942));
#96730=CARTESIAN_POINT('Ctrl Pts',(16.9369196023259,20.3300674755601,-7.18387582991034));
#96731=CARTESIAN_POINT('Ctrl Pts',(16.9464809059165,20.3452454095263,-7.18495543093504));
#96732=CARTESIAN_POINT('Ctrl Pts',(16.9502087417741,20.3510990788551,-7.18537201838789));
#96733=CARTESIAN_POINT('Ctrl Pts',(16.9574518113397,20.3623500853074,-7.18617318186877));
#96734=CARTESIAN_POINT('Ctrl Pts',(16.9609630201946,20.3677499104074,-7.18655790159666));
#96735=CARTESIAN_POINT('Ctrl Pts',(16.9690857741152,20.3801178700886,-7.1874396026037));
#96736=CARTESIAN_POINT('Ctrl Pts',(16.9737140585374,20.3870749237335,-7.18793595018522));
#96737=CARTESIAN_POINT('Ctrl Pts',(16.9861789676203,20.4055732481931,-7.18925686416091));
#96738=CARTESIAN_POINT('Ctrl Pts',(16.9940887662805,20.4170648901248,-7.19007866420648));
#96739=CARTESIAN_POINT('Ctrl Pts',(17.0590934138735,20.5095354016538,-7.196703466659));
#96740=CARTESIAN_POINT('Ctrl Pts',(17.1216989541706,20.5864981666697,-7.20228401728065));
#96741=CARTESIAN_POINT('Ctrl Pts',(17.2825129833919,20.7580561297849,-7.21524692116285));
#96742=CARTESIAN_POINT('Ctrl Pts',(17.3848991732431,20.8481077382555,-7.2224861209784));
#96743=CARTESIAN_POINT('Ctrl Pts',(17.5367053128296,20.9576517992095,-7.23286053549933));
#96744=CARTESIAN_POINT('Ctrl Pts',(17.5792667629144,20.9860767655471,-7.23573770530333));
#96745=CARTESIAN_POINT('Ctrl Pts',(17.6381061458833,21.0223609477645,-7.23973190087502));
#96746=CARTESIAN_POINT('Ctrl Pts',(17.6535182966053,21.0315963494275,-7.24077963095591));
#96747=CARTESIAN_POINT('Ctrl Pts',(17.6765035697603,21.0449751267277,-7.24234724049342));
#96748=CARTESIAN_POINT('Ctrl Pts',(17.6839878773896,21.0492703833593,-7.24285845665203));
#96749=CARTESIAN_POINT('Ctrl Pts',(17.6975880446207,21.0569653894606,-7.24378921449107));
#96750=CARTESIAN_POINT('Ctrl Pts',(17.7036949403113,21.0603808264406,-7.24420780397234));
#96751=CARTESIAN_POINT('Ctrl Pts',(17.7133464704446,21.0657160488772,-7.24487055778848));
#96752=CARTESIAN_POINT('Ctrl Pts',(17.7168799117131,21.0676561272182,-7.24511344546357));
#96753=CARTESIAN_POINT('Ctrl Pts',(17.7204279624832,21.0695910590746,-7.24535761187313));
#96754=CARTESIAN_POINT('Ctrl Pts',(17.7204370861311,21.0695960345749,-7.24535823973754));
#96755=CARTESIAN_POINT('Ctrl Pts',(17.7204553884822,21.0696060154246,-7.24535949925876));
#96756=CARTESIAN_POINT('Ctrl Pts',(17.7204645681256,21.0696110212857,-7.2453601309803));
#96757=CARTESIAN_POINT('Ctrl Pts',(17.7204829830544,21.0696210631736,-7.24536139825621));
#96758=CARTESIAN_POINT('Ctrl Pts',(17.7204922183432,21.0696260992012,-7.24536203381084));
#96759=CARTESIAN_POINT('Ctrl Pts',(17.7205107451867,21.0696362017592,-7.24536330879594));
#96760=CARTESIAN_POINT('Ctrl Pts',(17.7205200368771,21.0696412683626,-7.24536394823579));
#96761=CARTESIAN_POINT('Ctrl Pts',(17.7205386774589,21.0696514325787,-7.24536523105573));
#96762=CARTESIAN_POINT('Ctrl Pts',(17.720548025621,21.0696565297926,-7.24536587438567));
#96763=CARTESIAN_POINT('Ctrl Pts',(17.7205667794415,21.0696667553876,-7.24536716500621));
#96764=CARTESIAN_POINT('Ctrl Pts',(17.7205761849688,21.0696718836961,-7.24536781228781));
#96765=CARTESIAN_POINT('Ctrl Pts',(17.7205950533626,21.0696821713911,-7.24536911080094));
#96766=CARTESIAN_POINT('Ctrl Pts',(17.7206045166479,21.0696873310048,-7.24536976206131));
#96767=CARTESIAN_POINT('Ctrl Pts',(17.7206235007403,21.0696976814065,-7.2453710685446));
#96768=CARTESIAN_POINT('Ctrl Pts',(17.7206330220353,21.0697028724593,-7.24537172380113));
#96769=CARTESIAN_POINT('Ctrl Pts',(17.7206521232753,21.0697132863507,-7.24537303835446));
#96770=CARTESIAN_POINT('Ctrl Pts',(17.7206617026036,21.069718508852,-7.24537369760885));
#96771=CARTESIAN_POINT('Ctrl Pts',(17.720680920904,21.0697289861786,-7.24537502022636));
#96772=CARTESIAN_POINT('Ctrl Pts',(17.7206905589489,21.0697342404973,-7.2453756835257));
#96773=CARTESIAN_POINT('Ctrl Pts',(17.7207098940811,21.0697447811275,-7.24537701419181));
#96774=CARTESIAN_POINT('Ctrl Pts',(17.7207195919305,21.0697500678533,-7.24537768161106));
#96775=CARTESIAN_POINT('Ctrl Pts',(17.7207390087232,21.0697606526068,-7.24537901790538));
#96776=CARTESIAN_POINT('Ctrl Pts',(17.7207487852062,21.069765982001,-7.24537969074065));
#96777=CARTESIAN_POINT('Ctrl Pts',(17.7207683803763,21.0697766635939,-7.24538103931955));
#96778=CARTESIAN_POINT('Ctrl Pts',(17.7207781970177,21.0697820146773,-7.2453817149226));
#96779=CARTESIAN_POINT('Ctrl Pts',(17.7207978923608,21.069792750471,-7.24538307040406));
#96780=CARTESIAN_POINT('Ctrl Pts',(17.7208077698294,21.0697981345078,-7.24538375019762));
#96781=CARTESIAN_POINT('Ctrl Pts',(17.7208275871355,21.0698089363729,-7.24538511408145));
#96782=CARTESIAN_POINT('Ctrl Pts',(17.7208375254755,21.0698143533836,-7.24538579806865));
#96783=CARTESIAN_POINT('Ctrl Pts',(17.7208574977835,21.0698252393204,-7.24538717262884));
#96784=CARTESIAN_POINT('Ctrl Pts',(17.7208674811768,21.0698306806786,-7.24538785972093));
#96785=CARTESIAN_POINT('Ctrl Pts',(17.7238790919266,21.0714721006418,-7.2455951300355));
#96786=CARTESIAN_POINT('Ctrl Pts',(17.7268846133439,21.0731007715878,-7.24580218197887));
#96787=CARTESIAN_POINT('Ctrl Pts',(17.7339322768655,21.0768977972676,-7.24628815832281));
#96788=CARTESIAN_POINT('Ctrl Pts',(17.7379775178711,21.0790602920898,-7.24656745015073));
#96789=CARTESIAN_POINT('Ctrl Pts',(17.7504472573001,21.0856743160113,-7.24742938504249));
#96790=CARTESIAN_POINT('Ctrl Pts',(17.7588946710058,21.0900820573763,-7.24801468537723));
#96791=CARTESIAN_POINT('Ctrl Pts',(17.8729484600565,21.1486175538417,-7.25593299112372));
#96792=CARTESIAN_POINT('Ctrl Pts',(17.9828828037535,21.193823226574,-7.26373568158187));
#96793=CARTESIAN_POINT('Ctrl Pts',(18.2002237608063,21.2625159034343,-7.2787929182716));
#96794=CARTESIAN_POINT('Ctrl Pts',(18.3068407073153,21.2873364328448,-7.28601942828048));
#96795=CARTESIAN_POINT('Ctrl Pts',(18.4895868515106,21.3152002007156,-7.29790063593097));
#96796=CARTESIAN_POINT('Ctrl Pts',(18.5648324033085,21.3225825308915,-7.30265488511632));
#96797=CARTESIAN_POINT('Ctrl Pts',(18.6591777524235,21.3267615574797,-7.30844061745585));
#96798=CARTESIAN_POINT('Ctrl Pts',(18.6780469354016,21.3273446381995,-7.30958922427399));
#96799=CARTESIAN_POINT('Ctrl Pts',(18.7054876263538,21.3278253208458,-7.31124762150342));
#96800=CARTESIAN_POINT('Ctrl Pts',(18.7140542951703,21.327923372882,-7.31176366012941));
#96801=CARTESIAN_POINT('Ctrl Pts',(18.729072507239,21.3280040948256,-7.31266542426654));
#96802=CARTESIAN_POINT('Ctrl Pts',(18.7355237710752,21.3280092813316,-7.31305184993446));
#96803=CARTESIAN_POINT('Ctrl Pts',(18.748048802387,21.3279620975784,-7.31380030337932));
#96804=CARTESIAN_POINT('Ctrl Pts',(18.7541225124443,21.3279130773624,-7.31416243224764));
#96805=CARTESIAN_POINT('Ctrl Pts',(18.7686385535778,21.3277334406176,-7.31502600444102));
#96806=CARTESIAN_POINT('Ctrl Pts',(18.7770805211379,21.3275784558716,-7.31552668150358));
#96807=CARTESIAN_POINT('Ctrl Pts',(18.8075218680721,21.3268373853055,-7.31732671733205));
#96808=CARTESIAN_POINT('Ctrl Pts',(18.829513194303,21.325958767784,-7.31861693378437));
#96809=CARTESIAN_POINT('Ctrl Pts',(19.0377788224135,21.3143827802219,-7.33074962236542));
#96810=CARTESIAN_POINT('Ctrl Pts',(19.2218783332728,21.2794490197337,-7.34072459828343));
#96811=CARTESIAN_POINT('Ctrl Pts',(19.4744933246417,21.1958620347866,-7.3552331381672));
#96812=CARTESIAN_POINT('Ctrl Pts',(19.5484874192376,21.1666625306593,-7.35960649227267));
#96813=CARTESIAN_POINT('Ctrl Pts',(19.6532159466919,21.1183585244683,-7.36620478456722));
#96814=CARTESIAN_POINT('Ctrl Pts',(19.6853846945999,21.1025182569949,-7.36829054926929));
#96815=CARTESIAN_POINT('Ctrl Pts',(19.7237363476259,21.0824076379036,-7.37086770932076));
#96816=CARTESIAN_POINT('Ctrl Pts',(19.730320715458,21.0789104938978,-7.37131345092288));
#96817=CARTESIAN_POINT('Ctrl Pts',(19.7405472972989,21.0734094122539,-7.37201110339174));
#96818=CARTESIAN_POINT('Ctrl Pts',(19.7442023882848,21.0714293629624,-7.37226152169424));
#96819=CARTESIAN_POINT('Ctrl Pts',(19.7509821795613,21.0677307192622,-7.37272805501671));
#96820=CARTESIAN_POINT('Ctrl Pts',(19.7541083777658,21.0660149903441,-7.37294398730038));
#96821=CARTESIAN_POINT('Ctrl Pts',(19.7611816898355,21.0621097076624,-7.3734343888156));
#96822=CARTESIAN_POINT('Ctrl Pts',(19.7651261254746,21.0599154351204,-7.37370915667037));
#96823=CARTESIAN_POINT('Ctrl Pts',(19.7752974442387,21.0542145028935,-7.37442097812567));
#96824=CARTESIAN_POINT('Ctrl Pts',(19.7815135839026,21.0506889300288,-7.37485920308778));
#96825=CARTESIAN_POINT('Ctrl Pts',(19.819683820957,21.0287839562399,-7.37756931814198));
#96826=CARTESIAN_POINT('Ctrl Pts',(19.8511691369719,21.0096051848397,-7.37988789408028));
#96827=CARTESIAN_POINT('Ctrl Pts',(20.0254135707649,20.8971265814173,-7.39312559558253));
#96828=CARTESIAN_POINT('Ctrl Pts',(20.1569903203571,20.7876653327158,-7.40463270078883));
#96829=CARTESIAN_POINT('Ctrl Pts',(20.3393210104831,20.594362805871,-7.42189956824913));
#96830=CARTESIAN_POINT('Ctrl Pts',(20.3998925301422,20.5207917785657,-7.4279462252364));
#96831=CARTESIAN_POINT('Ctrl Pts',(20.4677517420899,20.426010473709,-7.43510637373632));
#96832=CARTESIAN_POINT('Ctrl Pts',(20.4799269402268,20.4084492583596,-7.43640876104));
#96833=CARTESIAN_POINT('Ctrl Pts',(20.4968529829134,20.3832284174491,-7.43824568559007));
#96834=CARTESIAN_POINT('Ctrl Pts',(20.5018237175899,20.3757185966945,-7.43878850992832));
#96835=CARTESIAN_POINT('Ctrl Pts',(20.5103134076187,20.3627127512104,-7.43972155808636));
#96836=CARTESIAN_POINT('Ctrl Pts',(20.5138551202073,20.35723179852,-7.44011263138249));
#96837=CARTESIAN_POINT('Ctrl Pts',(20.5205859737462,20.3467090940383,-7.44085940422798));
#96838=CARTESIAN_POINT('Ctrl Pts',(20.5237792519135,20.3416700749597,-7.44121525529247));
#96839=CARTESIAN_POINT('Ctrl Pts',(20.5320232807208,20.328538491335,-7.44213808373598));
#96840=CARTESIAN_POINT('Ctrl Pts',(20.5370407453188,20.320425109179,-7.44270382777409));
#96841=CARTESIAN_POINT('Ctrl Pts',(20.5539416676872,20.29267832489,-7.44462383532946));
#96842=CARTESIAN_POINT('Ctrl Pts',(20.5655609045994,20.27288529779,-7.44596844912395));
#96843=CARTESIAN_POINT('Ctrl Pts',(20.6634974616737,20.0996615221443,-7.45753208502275));
#96844=CARTESIAN_POINT('Ctrl Pts',(20.7306862124172,19.9362107264801,-7.46699461391883));
#96845=CARTESIAN_POINT('Ctrl Pts',(20.7995881303978,19.6827372782856,-7.4812880978165));
#96846=CARTESIAN_POINT('Ctrl Pts',(20.8171549941907,19.5978504647584,-7.48603083331034));
#96847=CARTESIAN_POINT('Ctrl Pts',(20.8348390110948,19.4747944306692,-7.49312956016931));
#96848=CARTESIAN_POINT('Ctrl Pts',(20.8392056194943,19.4373204709446,-7.49532097023031));
#96849=CARTESIAN_POINT('Ctrl Pts',(20.8432431692171,19.3922167140733,-7.49801528684611));
#96850=CARTESIAN_POINT('Ctrl Pts',(20.8438773414933,19.3846774144376,-7.49846755170978));
#96851=CARTESIAN_POINT('Ctrl Pts',(20.8447991883511,19.3729668715092,-7.4991732078071));
#96852=CARTESIAN_POINT('Ctrl Pts',(20.8451149494973,19.3687978147029,-7.49942505052457));
#96853=CARTESIAN_POINT('Ctrl Pts',(20.8456769821951,19.3610733960172,-7.49989286271574));
#96854=CARTESIAN_POINT('Ctrl Pts',(20.8459266269316,19.357518337416,-7.50010864075819));
#96855=CARTESIAN_POINT('Ctrl Pts',(20.8464699483691,19.3494911662168,-7.50059692363118));
#96856=CARTESIAN_POINT('Ctrl Pts',(20.8467583996017,19.3450187671209,-7.50086971606983));
#96857=CARTESIAN_POINT('Ctrl Pts',(20.8475658337507,19.3318486124493,-7.50167514161818));
#96858=CARTESIAN_POINT('Ctrl Pts',(20.848045315119,19.3231486529459,-7.50220990744066));
#96859=CARTESIAN_POINT('Ctrl Pts',(20.8510723984326,19.261274143636,-7.50603130835539));
#96860=CARTESIAN_POINT('Ctrl Pts',(20.851666915218,19.208027556936,-7.50941461509519));
#96861=CARTESIAN_POINT('Ctrl Pts',(20.8497710029055,19.136609620182,-7.51403157684536));
#96862=CARTESIAN_POINT('Ctrl Pts',(20.8490525361865,19.1184062218512,-7.51521531632575));
#96863=CARTESIAN_POINT('Ctrl Pts',(20.8455854336163,19.0522439970115,-7.51953830220375));
#96864=CARTESIAN_POINT('Ctrl Pts',(20.8414396610375,19.0043738706043,-7.52270509319466));
#96865=CARTESIAN_POINT('Ctrl Pts',(20.8225299999094,18.8481021103046,-7.53310328181739));
#96866=CARTESIAN_POINT('Ctrl Pts',(20.8009940056968,18.740689798978,-7.54033569773389));
#96867=CARTESIAN_POINT('Ctrl Pts',(20.7562719040651,18.5823977293319,-7.5509085411294));
#96868=CARTESIAN_POINT('Ctrl Pts',(20.7392273814701,18.5299798548734,-7.5543973484465));
#96869=CARTESIAN_POINT('Ctrl Pts',(20.7082838776819,18.4461021504203,-7.55995445463637));
#96870=CARTESIAN_POINT('Ctrl Pts',(20.6956311008092,18.4142132088306,-7.56206118425963));
#96871=CARTESIAN_POINT('Ctrl Pts',(20.6779792588378,18.3726978719752,-7.56479756475719));
#96872=CARTESIAN_POINT('Ctrl Pts',(20.6736739859594,18.3627838414531,-7.56545055379049));
#96873=CARTESIAN_POINT('Ctrl Pts',(20.6664969221183,18.3465971843096,-7.56651603476649));
#96874=CARTESIAN_POINT('Ctrl Pts',(20.6636701020753,18.3403049439217,-7.5669300560485));
#96875=CARTESIAN_POINT('Ctrl Pts',(20.6581378197626,18.3281498766367,-7.56772956918661));
#96876=CARTESIAN_POINT('Ctrl Pts',(20.6554361936147,18.3222853972975,-7.56811518736254));
#96877=CARTESIAN_POINT('Ctrl Pts',(20.649135079636,18.3087704782615,-7.56900361702094));
#96878=CARTESIAN_POINT('Ctrl Pts',(20.6455164912051,18.3011290255409,-7.56950576239384));
#96879=CARTESIAN_POINT('Ctrl Pts',(20.6356589069633,18.2806309267153,-7.57085240739178));
#96880=CARTESIAN_POINT('Ctrl Pts',(20.6293352837622,18.2678152948676,-7.5716939653678));
#96881=CARTESIAN_POINT('Ctrl Pts',(20.5701090635873,18.1507871592397,-7.57937783534059));
#96882=CARTESIAN_POINT('Ctrl Pts',(20.5087886474078,18.0510524646779,-7.58590326270512));
#96883=CARTESIAN_POINT('Ctrl Pts',(20.3430433535936,17.8256474079191,-7.60121970882826));
#96884=CARTESIAN_POINT('Ctrl Pts',(20.2317349114003,17.7060081278881,-7.60982722065062));
#96885=CARTESIAN_POINT('Ctrl Pts',(20.0832288320186,17.5793394470836,-7.62103684117124));
#96886=CARTESIAN_POINT('Ctrl Pts',(20.0581507781137,17.5589228043075,-7.62292306799144));
#96887=CARTESIAN_POINT('Ctrl Pts',(20.0269084398209,17.5346560594328,-7.62527854330196));
#96888=CARTESIAN_POINT('Ctrl Pts',(20.0211776913712,17.5302517058625,-7.62571083106226));
#96889=CARTESIAN_POINT('Ctrl Pts',(20.0121553637404,17.5233908229729,-7.62639196177655));
#96890=CARTESIAN_POINT('Ctrl Pts',(20.0088789361461,17.5209143318292,-7.62663942471207));
#96891=CARTESIAN_POINT('Ctrl Pts',(20.0027392654977,17.5163016676524,-7.62710339668077));
#96892=CARTESIAN_POINT('Ctrl Pts',(19.9998778149962,17.5141632022144,-7.62731974131291));
#96893=CARTESIAN_POINT('Ctrl Pts',(19.9933309874139,17.5092962976818,-7.62781495791823));
#96894=CARTESIAN_POINT('Ctrl Pts',(19.9896421621321,17.5065725928903,-7.62809415311311));
#96895=CARTESIAN_POINT('Ctrl Pts',(19.9782674078456,17.4982308227799,-7.62895549994657));
#96896=CARTESIAN_POINT('Ctrl Pts',(19.9705525307129,17.492652692943,-7.6295403037076));
#96897=CARTESIAN_POINT('Ctrl Pts',(19.8652496884133,17.4175913779459,-7.63752762654764));
#96898=CARTESIAN_POINT('Ctrl Pts',(19.7619835706889,17.3564694739561,-7.64540854906931));
#96899=CARTESIAN_POINT('Ctrl Pts',(19.5560347535918,17.2570785883419,-7.66051581876532));
#96900=CARTESIAN_POINT('Ctrl Pts',(19.4544369281335,17.2173791409806,-7.66771430848045));
#96901=CARTESIAN_POINT('Ctrl Pts',(19.2785324977121,17.1638581666769,-7.67952731461302));
#96902=CARTESIAN_POINT('Ctrl Pts',(19.2057218935698,17.1458641883269,-7.68424212820552));
#96903=CARTESIAN_POINT('Ctrl Pts',(19.1136428664124,17.1282341578661,-7.68998531474084));
#96904=CARTESIAN_POINT('Ctrl Pts',(19.0951362961006,17.124945621375,-7.69112888288112));
#96905=CARTESIAN_POINT('Ctrl Pts',(19.0681485823209,17.120519944509,-7.69278138706911));
#96906=CARTESIAN_POINT('Ctrl Pts',(19.0597008573032,17.1191871277819,-7.69329650913612));
#96907=CARTESIAN_POINT('Ctrl Pts',(19.0448691569094,17.1169391233765,-7.69419721569517));
#96908=CARTESIAN_POINT('Ctrl Pts',(19.0384886876958,17.116001854842,-7.69458349531606));
#96909=CARTESIAN_POINT('Ctrl Pts',(19.0260863014067,17.1142378443043,-7.69533206077629));
#96910=CARTESIAN_POINT('Ctrl Pts',(19.0200649169497,17.1134078543475,-7.69569444584988));
#96911=CARTESIAN_POINT('Ctrl Pts',(19.0056543965734,17.1114847084589,-7.69655925733277));
#96912=CARTESIAN_POINT('Ctrl Pts',(18.9972620770168,17.1104158782485,-7.69706091240715));
#96913=CARTESIAN_POINT('Ctrl Pts',(18.9669110287855,17.1067351758464,-7.69886816321529));
#96914=CARTESIAN_POINT('Ctrl Pts',(18.9449176328586,17.1044170313075,-7.7001645191002));
#96915=CARTESIAN_POINT('Ctrl Pts',(18.7380956070199,17.0858892411994,-7.71224140454963));
#96916=CARTESIAN_POINT('Ctrl Pts',(18.5519309717436,17.0936976127733,-7.72216589755605));
#96917=CARTESIAN_POINT('Ctrl Pts',(18.2613168852555,17.1445429407069,-7.73824897429961));
#96918=CARTESIAN_POINT('Ctrl Pts',(18.1551181761788,17.1717443709271,-7.7442837374116));
#96919=CARTESIAN_POINT('Ctrl Pts',(18.0403470630171,17.2108315624758,-7.75143990705116));
#96920=CARTESIAN_POINT('Ctrl Pts',(18.0292119362402,17.2147279878865,-7.75214107073281));
#96921=CARTESIAN_POINT('Ctrl Pts',(18.0134014140985,17.2204092047715,-7.75314722591709));
#96922=CARTESIAN_POINT('Ctrl Pts',(18.0086986522564,17.2221179044894,-7.75344784341923));
#96923=CARTESIAN_POINT('Ctrl Pts',(18.000594465435,17.2250950424322,-7.75396828200413));
#96924=CARTESIAN_POINT('Ctrl Pts',(17.9971901293249,17.2263556003775,-7.75418763399487));
#96925=CARTESIAN_POINT('Ctrl Pts',(17.9905875590405,17.2288197307567,-7.75461450451461));
#96926=CARTESIAN_POINT('Ctrl Pts',(17.9873889907919,17.2300222924787,-7.75482195672569));
#96927=CARTESIAN_POINT('Ctrl Pts',(17.9787494943091,17.233294369617,-7.75538404826525));
#96928=CARTESIAN_POINT('Ctrl Pts',(17.9733142149168,17.235378573378,-7.75573955416039));
#96929=CARTESIAN_POINT('Ctrl Pts',(17.9530711626596,17.243236863244,-7.75707044175574));
#96930=CARTESIAN_POINT('Ctrl Pts',(17.938320393228,17.2491550672372,-7.7580539427589));
#96931=CARTESIAN_POINT('Ctrl Pts',(17.8094457286009,17.3025537630838,-7.76675864107124));
#96932=CARTESIAN_POINT('Ctrl Pts',(17.6996273306895,17.3597747062125,-7.77493784328568));
#96933=CARTESIAN_POINT('Ctrl Pts',(17.4545089122284,17.5161443843451,-7.79415109477477));
#96934=CARTESIAN_POINT('Ctrl Pts',(17.324696423208,17.6224417721401,-7.80506921525835));
#96935=CARTESIAN_POINT('Ctrl Pts',(17.1939623569774,17.7582692823488,-7.81664814540657));
#96936=CARTESIAN_POINT('Ctrl Pts',(17.1794268297673,17.7738344596634,-7.81794607724562));
#96937=CARTESIAN_POINT('Ctrl Pts',(17.1590898627573,17.7962816739177,-7.81977786442136));
#96938=CARTESIAN_POINT('Ctrl Pts',(17.1530939813725,17.8029850687184,-7.82031994395172));
#96939=CARTESIAN_POINT('Ctrl Pts',(17.1428230046997,17.814616340643,-7.82125211385718));
#96940=CARTESIAN_POINT('Ctrl Pts',(17.1385276706298,17.8195261043826,-7.82164304948772));
#96941=CARTESIAN_POINT('Ctrl Pts',(17.1303462138068,17.8289655748825,-7.82238983293753));
#96942=CARTESIAN_POINT('Ctrl Pts',(17.1264564239609,17.8334920071229,-7.82274583095637));
#96943=CARTESIAN_POINT('Ctrl Pts',(17.1163900847981,17.8453066129552,-7.82366963190904));
#96944=CARTESIAN_POINT('Ctrl Pts',(17.1102435908696,17.8526203058302,-7.82423619624352));
#96945=CARTESIAN_POINT('Ctrl Pts',(17.0894465542836,17.8777095004407,-7.82616202302315));
#96946=CARTESIAN_POINT('Ctrl Pts',(17.0750363886521,17.8956827798896,-7.82751155488038));
#96947=CARTESIAN_POINT('Ctrl Pts',(16.9537660001987,18.0521032357074,-7.83901211222878));
#96948=CARTESIAN_POINT('Ctrl Pts',(16.8641494981791,18.203061196504,-7.848418175652));
#96949=CARTESIAN_POINT('Ctrl Pts',(16.7766288646635,18.403352548604,-7.86031011670247));
#96950=CARTESIAN_POINT('Ctrl Pts',(16.7603898995266,18.4438903486588,-7.86269366584045));
#96951=CARTESIAN_POINT('Ctrl Pts',(16.7454194594376,18.48488951688,-7.86510585860832));
#96952=CARTESIAN_POINT('',(16.6156461087368,19.2092594235966,-6.88905704663753));
#96953=CARTESIAN_POINT('Ctrl Pts',(16.743090251011,18.4840590306076,-7.64456001983877));
#96954=CARTESIAN_POINT('Ctrl Pts',(16.7690655518128,18.4111456296853,-7.63988948018787));
#96955=CARTESIAN_POINT('Ctrl Pts',(17.0725682250524,17.6922648295445,-7.59282700497648));
#96956=CARTESIAN_POINT('Ctrl Pts',(18.4531255372358,16.7235436104772,-7.50337259420462));
#96957=CARTESIAN_POINT('Ctrl Pts',(20.6735251555922,17.6284160608558,-7.3761967875232));
#96958=CARTESIAN_POINT('Ctrl Pts',(21.1145308242001,19.9852110491624,-7.24902098084175));
#96959=CARTESIAN_POINT('Ctrl Pts',(19.3715472140107,21.6317154528194,-7.12184517416032));
#96960=CARTESIAN_POINT('Ctrl Pts',(17.1752234436464,21.0898253692303,-7.00185719609225));
#96961=CARTESIAN_POINT('Ctrl Pts',(16.6208560614913,19.7934638448055,-6.92426115358465));
#96962=CARTESIAN_POINT('Ctrl Pts',(16.6156461087368,19.2092594235966,-6.88905704663753));
#96963=CARTESIAN_POINT('Ctrl Pts',(16.6170007608246,19.2092051933703,-6.88983560272607));
#96964=CARTESIAN_POINT('Ctrl Pts',(16.6170691234831,19.1285704923251,-6.88542652681705));
#96965=CARTESIAN_POINT('Ctrl Pts',(16.621744409621,19.0480107499138,-6.88096271700477));
#96966=CARTESIAN_POINT('Ctrl Pts',(16.6337263173979,18.944349549339,-6.8749294996215));
#96967=CARTESIAN_POINT('Ctrl Pts',(16.6368467594814,18.9208273159821,-6.87354087664655));
#96968=CARTESIAN_POINT('Ctrl Pts',(16.6412443064366,18.8914720729822,-6.87177780667558));
#96969=CARTESIAN_POINT('Ctrl Pts',(16.6421517369496,18.8855843710229,-6.87142267176195));
#96970=CARTESIAN_POINT('Ctrl Pts',(16.6437164847236,18.8757088423748,-6.87082432682732));
#96971=CARTESIAN_POINT('Ctrl Pts',(16.6443603995873,18.8717188858875,-6.87058184750745));
#96972=CARTESIAN_POINT('Ctrl Pts',(16.6455600505918,18.8644183406169,-6.87013679264496));
#96973=CARTESIAN_POINT('Ctrl Pts',(16.6461122450045,18.8611071720033,-6.86993441614739));
#96974=CARTESIAN_POINT('Ctrl Pts',(16.647268751021,18.8542725486385,-6.86951558516495));
#96975=CARTESIAN_POINT('Ctrl Pts',(16.6478741076568,18.8507493363769,-6.86929906988327));
#96976=CARTESIAN_POINT('Ctrl Pts',(16.6492807993464,18.8426847537831,-6.86880208190678));
#96977=CARTESIAN_POINT('Ctrl Pts',(16.6500880489582,18.8381444709462,-6.86852127706985));
#96978=CARTESIAN_POINT('Ctrl Pts',(16.6526310873336,18.8241077074899,-6.8676501046972));
#96979=CARTESIAN_POINT('Ctrl Pts',(16.6544169762281,18.8146205911576,-6.86705699836012));
#96980=CARTESIAN_POINT('Ctrl Pts',(16.6735179717447,18.7168347401309,-6.86090160543583));
#96981=CARTESIAN_POINT('Ctrl Pts',(16.6963792374528,18.6297226697183,-6.85506651331012));
#96982=CARTESIAN_POINT('Ctrl Pts',(16.7313173629578,18.5244202611044,-6.84777452238905));
#96983=CARTESIAN_POINT('Ctrl Pts',(16.7382219241471,18.5046012268794,-6.8463911615787));
#96984=CARTESIAN_POINT('Ctrl Pts',(16.7454194487812,18.4848895460645,-6.84500598950246));
#96985=CARTESIAN_POINT('Origin',(18.734,19.211,0.));
#96986=CARTESIAN_POINT('',(16.7454194503114,18.4848895418737,-6.04247203357104));
#96987=CARTESIAN_POINT('',(16.7454195730112,18.484889205839,-6.26710634208694));
#96988=CARTESIAN_POINT('',(16.7454194503191,18.4848895418526,0.));
#96989=CARTESIAN_POINT('Ctrl Pts',(16.7454195730112,18.484889205839,-6.26710634208694));
#96990=CARTESIAN_POINT('Ctrl Pts',(16.7157171128003,18.5662345480153,-6.27277683141834));
#96991=CARTESIAN_POINT('Ctrl Pts',(16.6910043038225,18.6494072568333,-6.27836337269697));
#96992=CARTESIAN_POINT('Ctrl Pts',(16.6614520778875,18.7771761929411,-6.28658111049015));
#96993=CARTESIAN_POINT('Ctrl Pts',(16.6528139479689,18.8207141214286,-6.28932034142043));
#96994=CARTESIAN_POINT('Ctrl Pts',(16.643614442751,18.8761611018695,-6.29273463347285));
#96995=CARTESIAN_POINT('Ctrl Pts',(16.6417764797029,18.8878442857266,-6.2934499418142));
#96996=CARTESIAN_POINT('Ctrl Pts',(16.6389885134331,18.9065880907435,-6.29459110135969));
#96997=CARTESIAN_POINT('Ctrl Pts',(16.6379760966145,18.9136390447423,-6.29501892187042));
#96998=CARTESIAN_POINT('Ctrl Pts',(16.6361227659987,18.9270264690196,-6.29582849659302));
#96999=CARTESIAN_POINT('Ctrl Pts',(16.6352749264759,18.9333618859301,-6.29621046570273));
#97000=CARTESIAN_POINT('Ctrl Pts',(16.633414069615,18.9477627967033,-6.2970761417738));
#97001=CARTESIAN_POINT('Ctrl Pts',(16.6324187831995,18.9558305109566,-6.29755928406061));
#97002=CARTESIAN_POINT('Ctrl Pts',(16.6299653952527,18.976706278146,-6.29880483450005));
#97003=CARTESIAN_POINT('Ctrl Pts',(16.6285777510808,18.9895223920608,-6.2995650214894));
#97004=CARTESIAN_POINT('Ctrl Pts',(16.6203967172453,19.0721247124333,-6.30443699776595));
#97005=CARTESIAN_POINT('Ctrl Pts',(16.6169563815465,19.142203345731,-6.30844165782057));
#97006=CARTESIAN_POINT('Ctrl Pts',(16.6171212273729,19.404716566235,-6.32314064332877));
#97007=CARTESIAN_POINT('Ctrl Pts',(16.6434647832249,19.5961655962577,-6.33317497168615));
#97008=CARTESIAN_POINT('Ctrl Pts',(16.7087052272871,19.8293426842463,-6.34683369412467));
#97009=CARTESIAN_POINT('Ctrl Pts',(16.7238020860671,19.8767853212513,-6.34969719296323));
#97010=CARTESIAN_POINT('Ctrl Pts',(16.7431845120058,19.9310025697894,-6.3531151035776));
#97011=CARTESIAN_POINT('Ctrl Pts',(16.745854488552,19.9383427175655,-6.35358097284039));
#97012=CARTESIAN_POINT('Ctrl Pts',(16.7501831752621,19.9500409657708,-6.35432872032372));
#97013=CARTESIAN_POINT('Ctrl Pts',(16.7518158006495,19.9544087315157,-6.35460908603248));
#97014=CARTESIAN_POINT('Ctrl Pts',(16.7547310332478,19.9621299809108,-6.35510686137764));
#97015=CARTESIAN_POINT('Ctrl Pts',(16.7560077573438,19.9654856385674,-6.35532391746722));
#97016=CARTESIAN_POINT('Ctrl Pts',(16.7587298594131,19.9725858335179,-6.35578473757404));
#97017=CARTESIAN_POINT('Ctrl Pts',(16.7601773291796,19.9763294543171,-6.3560286205799));
#97018=CARTESIAN_POINT('Ctrl Pts',(16.7641078966439,19.9864098411805,-6.35668773924526));
#97019=CARTESIAN_POINT('Ctrl Pts',(16.7666108960728,19.9927387232977,-6.35710414401619));
#97020=CARTESIAN_POINT('Ctrl Pts',(16.7791207440013,20.0239294846929,-6.35916870416381));
#97021=CARTESIAN_POINT('Ctrl Pts',(16.7895680738967,20.04861063857,-6.36084133192827));
#97022=CARTESIAN_POINT('Ctrl Pts',(16.8210382317118,20.1191931594763,-6.36572419259452));
#97023=CARTESIAN_POINT('Ctrl Pts',(16.8432373509301,20.1645478312475,-6.36898503169949));
#97024=CARTESIAN_POINT('Ctrl Pts',(16.9295817032383,20.3260626903425,-6.38094756479307));
#97025=CARTESIAN_POINT('Ctrl Pts',(17.0029893298191,20.4369262419257,-6.3898157700923));
#97026=CARTESIAN_POINT('Ctrl Pts',(17.1511163185503,20.6205484644966,-6.4051416947578));
#97027=CARTESIAN_POINT('Ctrl Pts',(17.2217357974137,20.6960623176748,-6.41168263632886));
#97028=CARTESIAN_POINT('Ctrl Pts',(17.307910781157,20.7756583472694,-6.41884328657374));
#97029=CARTESIAN_POINT('Ctrl Pts',(17.3183213353504,20.7850839041021,-6.41969609490092));
#97030=CARTESIAN_POINT('Ctrl Pts',(17.3350950524069,20.7999695466006,-6.42105098750275));
#97031=CARTESIAN_POINT('Ctrl Pts',(17.3413980605066,20.8054965078987,-6.42155587251278));
#97032=CARTESIAN_POINT('Ctrl Pts',(17.3526049402554,20.8152064172839,-6.4224461732826));
#97033=CARTESIAN_POINT('Ctrl Pts',(17.3574953667403,20.8194046556701,-6.42283222174498));
#97034=CARTESIAN_POINT('Ctrl Pts',(17.367682200866,20.8280691602798,-6.42363132400555));
#97035=CARTESIAN_POINT('Ctrl Pts',(17.3729815193615,20.8325318974578,-6.42404422991631));
#97036=CARTESIAN_POINT('Ctrl Pts',(17.3867089423316,20.8439775246914,-6.42510670644005));
#97037=CARTESIAN_POINT('Ctrl Pts',(17.3951695301738,20.8509212694798,-6.42575467924603));
#97038=CARTESIAN_POINT('Ctrl Pts',(17.4313068445597,20.8801136921761,-6.42849388356384));
#97039=CARTESIAN_POINT('Ctrl Pts',(17.4594881412675,20.9017305266963,-6.43055977652761));
#97040=CARTESIAN_POINT('Ctrl Pts',(17.5349317069356,20.9566416643685,-6.43592258394742));
#97041=CARTESIAN_POINT('Ctrl Pts',(17.5830376528115,20.9887277618309,-6.43917556783512));
#97042=CARTESIAN_POINT('Ctrl Pts',(17.7707936119587,21.1031382717155,-6.45137508646922));
#97043=CARTESIAN_POINT('Ctrl Pts',(17.918402403406,21.1712930695367,-6.45992612162854));
#97044=CARTESIAN_POINT('Ctrl Pts',(18.0929235931255,21.2287165275406,-6.47018706747939));
#97045=CARTESIAN_POINT('Ctrl Pts',(18.1136180628487,21.235175176664,-6.47140682939451));
#97046=CARTESIAN_POINT('Ctrl Pts',(18.1746823789171,21.2532086898565,-6.4750245016199));
#97047=CARTESIAN_POINT('Ctrl Pts',(18.2152992908394,21.2639007717696,-6.47745423736939));
#97048=CARTESIAN_POINT('Ctrl Pts',(18.2634493062217,21.2750558024442,-6.48039067042102));
#97049=CARTESIAN_POINT('Ctrl Pts',(18.2707032256743,21.2766961069424,-6.480834536319));
#97050=CARTESIAN_POINT('Ctrl Pts',(18.2824592935057,21.2792894302036,-6.48155651000256));
#97051=CARTESIAN_POINT('Ctrl Pts',(18.2869562422889,21.2802660666255,-6.48183329998524));
#97052=CARTESIAN_POINT('Ctrl Pts',(18.2949512390077,21.2819751225672,-6.48232655440146));
#97053=CARTESIAN_POINT('Ctrl Pts',(18.2984479937798,21.282713354323,-6.48254268280818));
#97054=CARTESIAN_POINT('Ctrl Pts',(18.305956854378,21.2842787671131,-6.48300765605414));
#97055=CARTESIAN_POINT('Ctrl Pts',(18.3099694368348,21.285103146307,-6.48325665137753));
#97056=CARTESIAN_POINT('Ctrl Pts',(18.3210209192156,21.2873402469347,-6.48394382674732));
#97057=CARTESIAN_POINT('Ctrl Pts',(18.3280645758112,21.2887288009247,-6.48438334857316));
#97058=CARTESIAN_POINT('Ctrl Pts',(18.3661876257942,21.2960429496807,-6.48677008586415));
#97059=CARTESIAN_POINT('Ctrl Pts',(18.3973880696127,21.3013067249018,-6.48875163643175));
#97060=CARTESIAN_POINT('Ctrl Pts',(18.5904538319102,21.3294442273624,-6.50113882603053));
#97061=CARTESIAN_POINT('Ctrl Pts',(18.7543963181856,21.3342040052771,-6.51214905143024));
#97062=CARTESIAN_POINT('Ctrl Pts',(19.033863009623,21.3099216097585,-6.53047401432928));
#97063=CARTESIAN_POINT('Ctrl Pts',(19.1494470995104,21.2901347497806,-6.53793075640742));
#97064=CARTESIAN_POINT('Ctrl Pts',(19.2766584604555,21.2573174411523,-6.54595261245501));
#97065=CARTESIAN_POINT('Ctrl Pts',(19.2904615824294,21.2536071080057,-6.54682078078264));
#97066=CARTESIAN_POINT('Ctrl Pts',(19.3123692542439,21.2474796831419,-6.5481953353323));
#97067=CARTESIAN_POINT('Ctrl Pts',(19.3204985392718,21.2451533769057,-6.54870465125274));
#97068=CARTESIAN_POINT('Ctrl Pts',(19.3348107027257,21.2409648249728,-6.54960009375852));
#97069=CARTESIAN_POINT('Ctrl Pts',(19.3409993664486,21.2391228911732,-6.54998687676749));
#97070=CARTESIAN_POINT('Ctrl Pts',(19.3537815742112,21.235254771121,-6.55078493332448));
#97071=CARTESIAN_POINT('Ctrl Pts',(19.3603738437984,21.2332246135568,-6.55119607164699));
#97072=CARTESIAN_POINT('Ctrl Pts',(19.3772687685316,21.2279311049686,-6.55224866142945));
#97073=CARTESIAN_POINT('Ctrl Pts',(19.3875566512589,21.2246209923689,-6.55288857227804));
#97074=CARTESIAN_POINT('Ctrl Pts',(19.4303800397828,21.2104798528851,-6.55554828537603));
#97075=CARTESIAN_POINT('Ctrl Pts',(19.4626763936725,21.1989375622901,-6.55754458038087));
#97076=CARTESIAN_POINT('Ctrl Pts',(19.5460742144948,21.1668265463782,-6.56268602732294));
#97077=CARTESIAN_POINT('Ctrl Pts',(19.5966794961533,21.1450389708372,-6.56579184308038));
#97078=CARTESIAN_POINT('Ctrl Pts',(19.7450263109169,21.0741869426091,-6.57493321228813));
#97079=CARTESIAN_POINT('Ctrl Pts',(19.8398773419618,21.019501030057,-6.580820026276));
#97080=CARTESIAN_POINT('Ctrl Pts',(19.9655515286581,20.9334453563047,-6.58911251296097));
#97081=CARTESIAN_POINT('Ctrl Pts',(20.0002738703543,20.9080820452341,-6.59146252736311));
#97082=CARTESIAN_POINT('Ctrl Pts',(20.0938178827419,20.8352818488065,-6.59802444682895));
#97083=CARTESIAN_POINT('Ctrl Pts',(20.1509039538893,20.7857307108622,-6.60229314793768));
#97084=CARTESIAN_POINT('Ctrl Pts',(20.2120398661685,20.7266441799308,-6.60733214094506));
#97085=CARTESIAN_POINT('Ctrl Pts',(20.2188216099872,20.7200009625788,-6.60789801861905));
#97086=CARTESIAN_POINT('Ctrl Pts',(20.2288085888273,20.710085474823,-6.60874207325033));
#97087=CARTESIAN_POINT('Ctrl Pts',(20.2320483621695,20.7068479474044,-6.60901758015181));
#97088=CARTESIAN_POINT('Ctrl Pts',(20.2377958807759,20.7010670141663,-6.6095094278243));
#97089=CARTESIAN_POINT('Ctrl Pts',(20.2403077206295,20.6985277504256,-6.60972543983958));
#97090=CARTESIAN_POINT('Ctrl Pts',(20.2456965520776,20.6930524388014,-6.61019116686551));
#97091=CARTESIAN_POINT('Ctrl Pts',(20.2485713798898,20.6901144078383,-6.61044103764561));
#97092=CARTESIAN_POINT('Ctrl Pts',(20.2564885481728,20.6819758975532,-6.61113304425547));
#97093=CARTESIAN_POINT('Ctrl Pts',(20.2615127264865,20.6767579395753,-6.61157655262607));
#97094=CARTESIAN_POINT('Ctrl Pts',(20.2889782033874,20.6479385614255,-6.6140246560007));
#97095=CARTESIAN_POINT('Ctrl Pts',(20.3108980520053,20.6238488617113,-6.61606566205947));
#97096=CARTESIAN_POINT('Ctrl Pts',(20.4389310805625,20.4764497057564,-6.6284723389654));
#97097=CARTESIAN_POINT('Ctrl Pts',(20.5310958998833,20.3417516120002,-6.63942741728655));
#97098=CARTESIAN_POINT('Ctrl Pts',(20.6613735314984,20.0944946623868,-6.6576827096116));
#97099=CARTESIAN_POINT('Ctrl Pts',(20.707181537781,19.9868182593872,-6.66512286385159));
#97100=CARTESIAN_POINT('Ctrl Pts',(20.7483642124681,19.8623294105699,-6.67312928268045));
#97101=CARTESIAN_POINT('Ctrl Pts',(20.752714704693,19.8487179143778,-6.67399725043238));
#97102=CARTESIAN_POINT('Ctrl Pts',(20.7594193994893,19.8269843620647,-6.67537154843671));
#97103=CARTESIAN_POINT('Ctrl Pts',(20.761863274943,19.81889063121,-6.67588080668667));
#97104=CARTESIAN_POINT('Ctrl Pts',(20.7660879240262,19.8045902274833,-6.67677618211034));
#97105=CARTESIAN_POINT('Ctrl Pts',(20.7678888987527,19.7983896816427,-6.67716295539817));
#97106=CARTESIAN_POINT('Ctrl Pts',(20.7715552247178,19.7855479002266,-6.67796102475101));
#97107=CARTESIAN_POINT('Ctrl Pts',(20.7734165419068,19.7789055852503,-6.67837218542874));
#97108=CARTESIAN_POINT('Ctrl Pts',(20.7781109614756,19.761832284549,-6.6794249004468));
#97109=CARTESIAN_POINT('Ctrl Pts',(20.7808967265067,19.7513884030041,-6.68006491345573));
#97110=CARTESIAN_POINT('Ctrl Pts',(20.7921897754932,19.7077099083396,-6.68272561932695));
#97111=CARTESIAN_POINT('Ctrl Pts',(20.7999688588139,19.674291221598,-6.68472278253884));
#97112=CARTESIAN_POINT('Ctrl Pts',(20.8181178131451,19.5867374798301,-6.68986697093002));
#97113=CARTESIAN_POINT('Ctrl Pts',(20.8271923872874,19.5323595930676,-6.69297460489443));
#97114=CARTESIAN_POINT('Ctrl Pts',(20.8479100000104,19.3692099757152,-6.70211914628175));
#97115=CARTESIAN_POINT('Ctrl Pts',(20.8532599550459,19.2598263349008,-6.70800732475787));
#97116=CARTESIAN_POINT('Ctrl Pts',(20.848826170494,19.1046941267489,-6.71645682681221));
#97117=CARTESIAN_POINT('Ctrl Pts',(20.8460283027936,19.0589247591212,-6.71896350962539));
#97118=CARTESIAN_POINT('Ctrl Pts',(20.8396436606771,18.9908615083874,-6.72275449525831));
#97119=CARTESIAN_POINT('Ctrl Pts',(20.83718274372,18.9684747894264,-6.72401170976417));
#97120=CARTESIAN_POINT('Ctrl Pts',(20.8337106790109,18.940941797381,-6.7255751164233));
#97121=CARTESIAN_POINT('Ctrl Pts',(20.8330369115128,18.9357539069997,-6.72587045500963));
#97122=CARTESIAN_POINT('Ctrl Pts',(20.8261932842122,18.8845460752896,-6.72879354682361));
#97123=CARTESIAN_POINT('Ctrl Pts',(20.8185306896726,18.8387420129144,-6.73147120945726));
#97124=CARTESIAN_POINT('Ctrl Pts',(20.8078579641483,18.7857226787476,-6.7346827493522));
#97125=CARTESIAN_POINT('Ctrl Pts',(20.8063058918322,18.7782229880204,-6.7351396651536));
#97126=CARTESIAN_POINT('Ctrl Pts',(20.8037527147901,18.7662146260185,-6.73587574119485));
#97127=CARTESIAN_POINT('Ctrl Pts',(20.8027774739496,18.7617004433096,-6.7361534623518));
#97128=CARTESIAN_POINT('Ctrl Pts',(20.8010190847327,18.7536883424341,-6.73664824517833));
#97129=CARTESIAN_POINT('Ctrl Pts',(20.8002418150537,18.7501891816113,-6.73686496796004));
#97130=CARTESIAN_POINT('Ctrl Pts',(20.7985697843028,18.7427512200483,-6.73732701225702));
#97131=CARTESIAN_POINT('Ctrl Pts',(20.797672650753,18.7388130623515,-6.73757246254138));
#97132=CARTESIAN_POINT('Ctrl Pts',(20.7952079244809,18.7281348237989,-6.73824015774943));
#97133=CARTESIAN_POINT('Ctrl Pts',(20.7936185610992,18.7213998916957,-6.73866362349529));
#97134=CARTESIAN_POINT('Ctrl Pts',(20.7853877115994,18.6872710681241,-6.74082096752433));
#97135=CARTESIAN_POINT('Ctrl Pts',(20.7782329354768,18.6600053871329,-6.74258198050917));
#97136=CARTESIAN_POINT('Ctrl Pts',(20.7556732807536,18.5805330752112,-6.74780920330726));
#97137=CARTESIAN_POINT('Ctrl Pts',(20.7387974357248,18.5287699578381,-6.75133417465667));
#97138=CARTESIAN_POINT('Ctrl Pts',(20.6713613069466,18.3461326208481,-6.76407932120529));
#97139=CARTESIAN_POINT('Ctrl Pts',(20.6098122617615,18.2196888925553,-6.77345467276722));
#97140=CARTESIAN_POINT('Ctrl Pts',(20.488640376356,18.0230836128615,-6.78836844067434));
#97141=CARTESIAN_POINT('Ctrl Pts',(20.4361602898219,17.9490323646912,-6.79408348275205));
#97142=CARTESIAN_POINT('Ctrl Pts',(20.3704427794626,17.867894412056,-6.80045431513944));
#97143=CARTESIAN_POINT('Ctrl Pts',(20.3616955804012,17.8573070132729,-6.80128804321739));
#97144=CARTESIAN_POINT('Ctrl Pts',(20.3475024048885,17.8404644303002,-6.80261846712928));
#97145=CARTESIAN_POINT('Ctrl Pts',(20.3421217297589,17.8341549601622,-6.80311780715638));
#97146=CARTESIAN_POINT('Ctrl Pts',(20.332502297046,17.8230083693917,-6.80400171080897));
#97147=CARTESIAN_POINT('Ctrl Pts',(20.3282783324153,17.8181586736077,-6.80438687758631));
#97148=CARTESIAN_POINT('Ctrl Pts',(20.3194315792848,17.8080943482046,-6.80518747776021));
#97149=CARTESIAN_POINT('Ctrl Pts',(20.3148050051731,17.80288313772,-6.80560274676184));
#97150=CARTESIAN_POINT('Ctrl Pts',(20.3027233509827,17.7894093794559,-6.80667839989021));
#97151=CARTESIAN_POINT('Ctrl Pts',(20.2952286401199,17.7811825344619,-6.80733710883089));
#97152=CARTESIAN_POINT('Ctrl Pts',(20.2624018629158,17.7457148782648,-6.81018592005663));
#97153=CARTESIAN_POINT('Ctrl Pts',(20.2364182363267,17.7190843072423,-6.81234803407614));
#97154=CARTESIAN_POINT('Ctrl Pts',(20.1655286855355,17.6501611737876,-6.81802236803161));
#97155=CARTESIAN_POINT('Ctrl Pts',(20.1194528596114,17.6091218999448,-6.82148366464681));
#97156=CARTESIAN_POINT('Ctrl Pts',(19.9571443547057,17.4768052867368,-6.83306940748254));
#97157=CARTESIAN_POINT('Ctrl Pts',(19.8331917225542,17.3957072764406,-6.84090300188289));
#97158=CARTESIAN_POINT('Ctrl Pts',(19.6393241600402,17.2960551869303,-6.85300994561398));
#97159=CARTESIAN_POINT('Ctrl Pts',(19.5752822611494,17.2670690594853,-6.85699439089739));
#97160=CARTESIAN_POINT('Ctrl Pts',(19.5012184820893,17.2378927087841,-6.86171342787288));
#97161=CARTESIAN_POINT('Ctrl Pts',(19.4924887560628,17.2345204575932,-6.86227136346605));
#97162=CARTESIAN_POINT('Ctrl Pts',(19.479478689503,17.2295936160018,-6.86310581070273));
#97163=CARTESIAN_POINT('Ctrl Pts',(19.4752150921646,17.2279947248406,-6.86337973981385));
#97164=CARTESIAN_POINT('Ctrl Pts',(19.4676002881612,17.2251670871743,-6.86386986829252));
#97165=CARTESIAN_POINT('Ctrl Pts',(19.464251101507,17.223933048699,-6.8640857478525));
#97166=CARTESIAN_POINT('Ctrl Pts',(19.4570211516786,17.2212898553458,-6.8645524503365));
#97167=CARTESIAN_POINT('Ctrl Pts',(19.4531394379694,17.2198836011928,-6.8648034357204));
#97168=CARTESIAN_POINT('Ctrl Pts',(19.4423586530324,17.2160136125355,-6.86550160666222));
#97169=CARTESIAN_POINT('Ctrl Pts',(19.4354509463233,17.2135743483709,-6.86595020445473));
#97170=CARTESIAN_POINT('Ctrl Pts',(19.3966033626951,17.2000827722967,-6.86847947658194));
#97171=CARTESIAN_POINT('Ctrl Pts',(19.3644169640888,17.1897614032853,-6.87059940516158));
#97172=CARTESIAN_POINT('Ctrl Pts',(19.2627751015612,17.1598312027444,-6.87734018874641));
#97173=CARTESIAN_POINT('Ctrl Pts',(19.1925582436769,17.1430011032718,-6.88206224799451));
#97174=CARTESIAN_POINT('Ctrl Pts',(19.1178327585342,17.1290835051586,-6.88707254751238));
#97175=CARTESIAN_POINT('Ctrl Pts',(19.1140388472069,17.1283876134826,-6.88732689190765));
#97176=CARTESIAN_POINT('Ctrl Pts',(18.9198653551403,17.0933199307972,-6.90034199432428));
#97177=CARTESIAN_POINT('Ctrl Pts',(18.725624994819,17.0851881656656,-6.91312367423729));
#97178=CARTESIAN_POINT('Ctrl Pts',(18.5118451743411,17.1055817086332,-6.92631837047566));
#97179=CARTESIAN_POINT('Ctrl Pts',(18.4907599493683,17.107913392808,-6.92761176153798));
#97180=CARTESIAN_POINT('Ctrl Pts',(18.461464000176,17.1115995505289,-6.92939820220442));
#97181=CARTESIAN_POINT('Ctrl Pts',(18.4532213852937,17.112686036112,-6.92989965952864));
#97182=CARTESIAN_POINT('Ctrl Pts',(18.439001869435,17.1146456444008,-6.93076277146269));
#97183=CARTESIAN_POINT('Ctrl Pts',(18.4330219560837,17.1154958364316,-6.93112514639025));
#97184=CARTESIAN_POINT('Ctrl Pts',(18.4206434725494,17.1173098233883,-6.93187405227898));
#97185=CARTESIAN_POINT('Ctrl Pts',(18.4142455115715,17.1182773863933,-6.93226045977063));
#97186=CARTESIAN_POINT('Ctrl Pts',(18.3992670317528,17.1206128745989,-6.93316356009079));
#97187=CARTESIAN_POINT('Ctrl Pts',(18.3906902582332,17.1220043277417,-6.93367950166247));
#97188=CARTESIAN_POINT('Ctrl Pts',(18.3628466393357,17.1266976499274,-6.93535079193471));
#97189=CARTESIAN_POINT('Ctrl Pts',(18.3436165531952,17.1302136327904,-6.93649934323863));
#97190=CARTESIAN_POINT('Ctrl Pts',(18.2453589231027,17.1495889630137,-6.9423423322874));
#97191=CARTESIAN_POINT('Ctrl Pts',(18.1672306245918,17.1696866760889,-6.94689956594685));
#97192=CARTESIAN_POINT('Ctrl Pts',(17.9590495531097,17.2361177755839,-6.95901426384232));
#97193=CARTESIAN_POINT('Ctrl Pts',(17.8320833022347,17.2907778884386,-6.96635672375421));
#97194=CARTESIAN_POINT('Ctrl Pts',(17.6378519725247,17.3979384419581,-6.97858082056443));
#97195=CARTESIAN_POINT('Ctrl Pts',(17.5668516874556,17.4428104892378,-6.98329659776018));
#97196=CARTESIAN_POINT('Ctrl Pts',(17.4909173473504,17.4973703412839,-6.9888371237247));
#97197=CARTESIAN_POINT('Ctrl Pts',(17.4831624783123,17.5030226655329,-6.98940904968154));
#97198=CARTESIAN_POINT('Ctrl Pts',(17.4717473791631,17.5114622734323,-6.99026041382681));
#97199=CARTESIAN_POINT('Ctrl Pts',(17.4680572509929,17.5142091707707,-6.99053711437982));
#97200=CARTESIAN_POINT('Ctrl Pts',(17.4616350699228,17.5190223941911,-6.99102132398669));
#97201=CARTESIAN_POINT('Ctrl Pts',(17.4588990429345,17.5210833502882,-6.99122845620957));
#97202=CARTESIAN_POINT('Ctrl Pts',(17.4530089302522,17.5255426202666,-6.99167621348503));
#97203=CARTESIAN_POINT('Ctrl Pts',(17.4498566198019,17.5279431149931,-6.99191698836922));
#97204=CARTESIAN_POINT('Ctrl Pts',(17.4415027435178,17.5343417510787,-6.99255805600139));
#97205=CARTESIAN_POINT('Ctrl Pts',(17.43631304118,17.5383552092597,-6.9929594065589));
#97206=CARTESIAN_POINT('Ctrl Pts',(17.4247881020536,17.547353945514,-6.99385746926857));
#97207=CARTESIAN_POINT('Ctrl Pts',(17.4184625488946,17.5523513939098,-6.99435498162914));
#97208=CARTESIAN_POINT('Ctrl Pts',(17.3994038955279,17.5675861227047,-6.99586756640451));
#97209=CARTESIAN_POINT('Ctrl Pts',(17.3867609144634,17.5779345554961,-6.99688951071415));
#97210=CARTESIAN_POINT('Ctrl Pts',(17.3401742285271,17.6169754966851,-7.00072079354399));
#97211=CARTESIAN_POINT('Ctrl Pts',(17.307018604272,17.6465870132565,-7.00357916107475));
#97212=CARTESIAN_POINT('Ctrl Pts',(17.226167502462,17.7235054878837,-7.01083888461658));
#97213=CARTESIAN_POINT('Ctrl Pts',(17.1797448443081,17.7720805639972,-7.01527737022366));
#97214=CARTESIAN_POINT('Ctrl Pts',(17.02753038308,17.947328282661,-7.03061698230959));
#97215=CARTESIAN_POINT('Ctrl Pts',(16.9342592505177,18.0841203921432,-7.04140633576255));
#97216=CARTESIAN_POINT('Ctrl Pts',(16.846879536144,18.2513007538768,-7.0530243892142));
#97217=CARTESIAN_POINT('Ctrl Pts',(16.8362948863819,18.2724044211339,-7.05446608172364));
#97218=CARTESIAN_POINT('Ctrl Pts',(16.8218844196206,18.3023768133364,-7.05647961300132));
#97219=CARTESIAN_POINT('Ctrl Pts',(16.8177631848946,18.3111008049072,-7.05706168934745));
#97220=CARTESIAN_POINT('Ctrl Pts',(16.8111821268346,18.3252820697487,-7.05800151106406));
#97221=CARTESIAN_POINT('Ctrl Pts',(16.8086855895395,18.330722062443,-7.05836052248939));
#97222=CARTESIAN_POINT('Ctrl Pts',(16.8035223705421,18.3420998394459,-7.05910828502606));
#97223=CARTESIAN_POINT('Ctrl Pts',(16.8008599314519,18.3480394889209,-7.05949688706339));
#97224=CARTESIAN_POINT('Ctrl Pts',(16.7946166550279,18.3621415395365,-7.06041540283663));
#97225=CARTESIAN_POINT('Ctrl Pts',(16.7910598711285,18.3703145035281,-7.06094448868439));
#97226=CARTESIAN_POINT('Ctrl Pts',(16.7793656291721,18.3976568086257,-7.06270391232643));
#97227=CARTESIAN_POINT('Ctrl Pts',(16.771459252064,18.4169241038271,-7.0639263982704));
#97228=CARTESIAN_POINT('Ctrl Pts',(16.7574991989216,18.4524265643442,-7.06614908213932));
#97229=CARTESIAN_POINT('Ctrl Pts',(16.7513592056384,18.4686224831075,-7.0671518274129));
#97230=CARTESIAN_POINT('Ctrl Pts',(16.7454194586292,18.4848895190942,-7.06814843723424));
#97231=CARTESIAN_POINT('Ctrl Pts',(16.7454194487812,18.4848895460645,-6.84500598950246));
#97232=CARTESIAN_POINT('Ctrl Pts',(16.7542717826021,18.4606458806915,-6.84330234745308));
#97233=CARTESIAN_POINT('Ctrl Pts',(16.7635672791046,18.4365646067694,-6.841595978446));
#97234=CARTESIAN_POINT('Ctrl Pts',(16.7883633738557,18.3756663207375,-6.83725152870356));
#97235=CARTESIAN_POINT('Ctrl Pts',(16.8044693734147,18.3391078640125,-6.83461588640926));
#97236=CARTESIAN_POINT('Ctrl Pts',(16.8668107437039,18.2078026951508,-6.82507743024927));
#97237=CARTESIAN_POINT('Ctrl Pts',(16.9190749575734,18.1160785924445,-6.81828421870596));
#97238=CARTESIAN_POINT('Ctrl Pts',(16.997360786519,17.9998107107914,-6.80956858496383));
#97239=CARTESIAN_POINT('Ctrl Pts',(17.017465563447,17.9714819466072,-6.8074349426178));
#97240=CARTESIAN_POINT('Ctrl Pts',(17.0447590019611,17.9349624880055,-6.80466927237634));
#97241=CARTESIAN_POINT('Ctrl Pts',(17.0513256322042,17.9263156573252,-6.80401327697482));
#97242=CARTESIAN_POINT('Ctrl Pts',(17.0621791624435,17.9122499016628,-6.80294414765039));
#97243=CARTESIAN_POINT('Ctrl Pts',(17.0664265223505,17.9068008475623,-6.80252946412771));
#97244=CARTESIAN_POINT('Ctrl Pts',(17.0746921769782,17.8963030071988,-6.80172953693702));
#97245=CARTESIAN_POINT('Ctrl Pts',(17.0787070239505,17.8912516151607,-6.80134416241328));
#97246=CARTESIAN_POINT('Ctrl Pts',(17.0880193242055,17.8796444299269,-6.80045752546651));
#97247=CARTESIAN_POINT('Ctrl Pts',(17.0933329815551,17.8731017315299,-6.79995692052343));
#97248=CARTESIAN_POINT('Ctrl Pts',(17.1077031384188,17.8556221388518,-6.79861712840315));
#97249=CARTESIAN_POINT('Ctrl Pts',(17.1168309339031,17.8447442205895,-6.79778083566769));
#97250=CARTESIAN_POINT('Ctrl Pts',(17.2242910857525,17.7192660218938,-6.78810147157151));
#97251=CARTESIAN_POINT('Ctrl Pts',(17.3345065385012,17.6154068130451,-6.77981373551478));
#97252=CARTESIAN_POINT('Ctrl Pts',(17.5448992440378,17.4558646820692,-6.76546513667802));
#97253=CARTESIAN_POINT('Ctrl Pts',(17.6402645547854,17.3949054109157,-6.75937827347752));
#97254=CARTESIAN_POINT('Ctrl Pts',(17.7804115104198,17.320378466526,-6.75039410020573));
#97255=CARTESIAN_POINT('Ctrl Pts',(17.8214750746974,17.3002204776161,-6.74775612581664));
#97256=CARTESIAN_POINT('Ctrl Pts',(17.8709182998608,17.2779062333554,-6.74453601841656));
#97257=CARTESIAN_POINT('Ctrl Pts',(17.8787018428705,17.2744498228436,-6.74402783233774));
#97258=CARTESIAN_POINT('Ctrl Pts',(17.8905418444945,17.2692773788094,-6.74325257622915));
#97259=CARTESIAN_POINT('Ctrl Pts',(17.8945832588591,17.2675268379475,-6.74298756255724));
#97260=CARTESIAN_POINT('Ctrl Pts',(17.9019055365098,17.2643822894027,-6.74250664980463));
#97261=CARTESIAN_POINT('Ctrl Pts',(17.9051844790447,17.2629839478799,-6.74229101863273));
#97262=CARTESIAN_POINT('Ctrl Pts',(17.9123080012485,17.2599672841148,-6.74182194653694));
#97263=CARTESIAN_POINT('Ctrl Pts',(17.9161537854684,17.2583520624674,-6.74156832750422));
#97264=CARTESIAN_POINT('Ctrl Pts',(17.9267613282122,17.2539337502809,-6.74086779275596));
#97265=CARTESIAN_POINT('Ctrl Pts',(17.933532815508,17.2511543780254,-6.74041948361966));
#97266=CARTESIAN_POINT('Ctrl Pts',(17.9681041072299,17.2371735674588,-6.73812552826431));
#97267=CARTESIAN_POINT('Ctrl Pts',(17.9961236412471,17.2265288938429,-6.7362494315757));
#97268=CARTESIAN_POINT('Ctrl Pts',(18.1901404732436,17.1574983883093,-6.72318893195346));
#97269=CARTESIAN_POINT('Ctrl Pts',(18.3626269434429,17.1194129446676,-6.71129873582195));
#97270=CARTESIAN_POINT('Ctrl Pts',(18.6346556991437,17.0940979638633,-6.69352822761822));
#97271=CARTESIAN_POINT('Ctrl Pts',(18.7319873364915,17.0917680736615,-6.687345065227));
#97272=CARTESIAN_POINT('Ctrl Pts',(18.8507355155976,17.0971104927864,-6.68004189407997));
#97273=CARTESIAN_POINT('Ctrl Pts',(18.872308998039,17.0984123202289,-6.67872443613411));
#97274=CARTESIAN_POINT('Ctrl Pts',(18.9028802793707,17.1007274360927,-6.67687014940629));
#97275=CARTESIAN_POINT('Ctrl Pts',(18.9118967832209,17.1014683976694,-6.67632481908893));
#97276=CARTESIAN_POINT('Ctrl Pts',(18.9274159536034,17.1028439454771,-6.67538881309296));
#97277=CARTESIAN_POINT('Ctrl Pts',(18.9339208869162,17.1034508732203,-6.67499727370422));
#97278=CARTESIAN_POINT('Ctrl Pts',(18.9463517558567,17.1046687772882,-6.67425052366811));
#97279=CARTESIAN_POINT('Ctrl Pts',(18.9522781159087,17.1052746728933,-6.67389515711057));
#97280=CARTESIAN_POINT('Ctrl Pts',(18.9676413680116,17.1069109273403,-6.67297554674825));
#97281=CARTESIAN_POINT('Ctrl Pts',(18.9770740948524,17.107979766287,-6.67241251892353));
#97282=CARTESIAN_POINT('Ctrl Pts',(19.0090051611747,17.1118156396605,-6.67051175500974));
#97283=CARTESIAN_POINT('Ctrl Pts',(19.0314666218217,17.1148806129644,-6.66918340357585));
#97284=CARTESIAN_POINT('Ctrl Pts',(19.2313636942161,17.1454355377504,-6.65742898485418));
#97285=CARTESIAN_POINT('Ctrl Pts',(19.404676806609,17.195032170277,-6.64779521464117));
#97286=CARTESIAN_POINT('Ctrl Pts',(19.6470153661258,17.2991475469224,-6.63343394423946));
#97287=CARTESIAN_POINT('Ctrl Pts',(19.7223109119337,17.336962601843,-6.62881653874044));
#97288=CARTESIAN_POINT('Ctrl Pts',(19.8272525208583,17.3977530694884,-6.62188710606429));
#97289=CARTESIAN_POINT('Ctrl Pts',(19.8588597232794,17.4171896058946,-6.61973081920961));
#97290=CARTESIAN_POINT('Ctrl Pts',(19.8962461114954,17.4415566759158,-6.61707543990428));
#97291=CARTESIAN_POINT('Ctrl Pts',(19.9025324118179,17.4457018100329,-6.61662530105815));
#97292=CARTESIAN_POINT('Ctrl Pts',(19.9122680213522,17.4521961776536,-6.61592225292707));
#97293=CARTESIAN_POINT('Ctrl Pts',(19.915732796055,17.4545222706566,-6.61567087382351));
#97294=CARTESIAN_POINT('Ctrl Pts',(19.9221442361277,17.4588541783392,-6.61520348087342));
#97295=CARTESIAN_POINT('Ctrl Pts',(19.9250927217109,17.46085719614,-6.61498765563757));
#97296=CARTESIAN_POINT('Ctrl Pts',(19.9317454213994,17.4654012249909,-6.6144986967956));
#97297=CARTESIAN_POINT('Ctrl Pts',(19.935446594759,17.4679465708481,-6.61422527205207));
#97298=CARTESIAN_POINT('Ctrl Pts',(19.9463423611838,17.4754909242637,-6.61341628429759));
#97299=CARTESIAN_POINT('Ctrl Pts',(19.9535139529155,17.4805227637334,-6.61287856085702));
#97300=CARTESIAN_POINT('Ctrl Pts',(20.0049966928034,17.5171238217646,-6.60898162470858));
#97301=CARTESIAN_POINT('Ctrl Pts',(20.0481037410525,17.5503436940706,-6.60552146289336));
#97302=CARTESIAN_POINT('Ctrl Pts',(20.2180186132341,17.6920472974389,-6.59121261856002));
#97303=CARTESIAN_POINT('Ctrl Pts',(20.3330781890264,17.8136866714715,-6.57998094787372));
#97304=CARTESIAN_POINT('Ctrl Pts',(20.4685097855369,17.9957749917055,-6.56533809923714));
#97305=CARTESIAN_POINT('Ctrl Pts',(20.5022877663718,18.0454720353527,-6.56152228729835));
#97306=CARTESIAN_POINT('Ctrl Pts',(20.5531251358018,18.1275771059215,-6.55550870807867));
#97307=CARTESIAN_POINT('Ctrl Pts',(20.5715361753906,18.1591052849395,-6.55326417240459));
#97308=CARTESIAN_POINT('Ctrl Pts',(20.594449000166,18.2007818531165,-6.5503782671967));
#97309=CARTESIAN_POINT('Ctrl Pts',(20.5996985063427,18.2105099814582,-6.54971025202415));
#97310=CARTESIAN_POINT('Ctrl Pts',(20.6081250907205,18.2264226922063,-6.54862653089586));
#97311=CARTESIAN_POINT('Ctrl Pts',(20.611348271691,18.232582502577,-6.54820919337355));
#97312=CARTESIAN_POINT('Ctrl Pts',(20.6174971544572,18.2444758668491,-6.54740752543332));
#97313=CARTESIAN_POINT('Ctrl Pts',(20.6204271601951,18.2502070974958,-6.54702304632916));
#97314=CARTESIAN_POINT('Ctrl Pts',(20.6270881511519,18.2633842489653,-6.54614320696507));
#97315=CARTESIAN_POINT('Ctrl Pts',(20.630801443708,18.2708390319669,-6.54564847142312));
#97316=CARTESIAN_POINT('Ctrl Pts',(20.6405752572889,18.2907545002039,-6.54433468192988));
#97317=CARTESIAN_POINT('Ctrl Pts',(20.6465576615999,18.3032532311985,-6.54351834672962));
#97318=CARTESIAN_POINT('Ctrl Pts',(20.6927450726799,18.4022341383204,-6.53711580671033));
#97319=CARTESIAN_POINT('Ctrl Pts',(20.7271898048286,18.4912902204123,-6.5317346905494));
#97320=CARTESIAN_POINT('Ctrl Pts',(20.7967396199892,18.7149466265282,-6.51880067871141));
#97321=CARTESIAN_POINT('Ctrl Pts',(20.8248222289333,18.8512449395767,-6.51141816111785));
#97322=CARTESIAN_POINT('Ctrl Pts',(20.8447997532398,19.040965656807,-6.50085289854419));
#97323=CARTESIAN_POINT('Ctrl Pts',(20.8483359065685,19.0928043126347,-6.49793397667051));
#97324=CARTESIAN_POINT('Ctrl Pts',(20.8508174969009,19.1720241999118,-6.49335590827038));
#97325=CARTESIAN_POINT('Ctrl Pts',(20.8511441638215,19.1993441915293,-6.49175579928983));
#97326=CARTESIAN_POINT('Ctrl Pts',(20.8508913970721,19.2335106195167,-6.48971962733981));
#97327=CARTESIAN_POINT('Ctrl Pts',(20.8508074859012,19.2403594906786,-6.48930970074442));
#97328=CARTESIAN_POINT('Ctrl Pts',(20.8506215274288,19.2512305543346,-6.48865606439309));
#97329=CARTESIAN_POINT('Ctrl Pts',(20.8505412462194,19.2552531389646,-6.4884135560312));
#97330=CARTESIAN_POINT('Ctrl Pts',(20.8503676775473,19.2628625857655,-6.48795354559231));
#97331=CARTESIAN_POINT('Ctrl Pts',(20.850276738111,19.2664494487498,-6.48773617604299));
#97332=CARTESIAN_POINT('Ctrl Pts',(20.8500471308375,19.2746798377041,-6.4872361893731));
#97333=CARTESIAN_POINT('Ctrl Pts',(20.8499022964849,19.2793231471537,-6.48695323076861));
#97334=CARTESIAN_POINT('Ctrl Pts',(20.8494750150797,19.2917127346766,-6.48619593355269));
#97335=CARTESIAN_POINT('Ctrl Pts',(20.8491653073926,19.2994579174424,-6.4857201318927));
#97336=CARTESIAN_POINT('Ctrl Pts',(20.8466146950027,19.3555286809475,-6.48225915387325));
#97337=CARTESIAN_POINT('Ctrl Pts',(20.8427605623458,19.4037627607391,-6.47919366098141));
#97338=CARTESIAN_POINT('Ctrl Pts',(20.8363724581257,19.4595552149184,-6.47557653274864));
#97339=CARTESIAN_POINT('Ctrl Pts',(20.835443900775,19.4672872938789,-6.47507364404561));
#97340=CARTESIAN_POINT('Ctrl Pts',(20.8135613229882,19.6413832073111,-6.46371677511084));
#97341=CARTESIAN_POINT('Ctrl Pts',(20.7729588608621,19.8046828863509,-6.45243043119019));
#97342=CARTESIAN_POINT('Ctrl Pts',(20.6927142930439,20.016336967326,-6.4378402413365));
#97343=CARTESIAN_POINT('Ctrl Pts',(20.669649319687,20.0702973883572,-6.43411711356651));
#97344=CARTESIAN_POINT('Ctrl Pts',(20.6289065285392,20.1556196158572,-6.42823223849908));
#97345=CARTESIAN_POINT('Ctrl Pts',(20.6126202391513,20.1876080150737,-6.42602616881911));
#97346=CARTESIAN_POINT('Ctrl Pts',(20.5902955315046,20.2288293608739,-6.42318188884288));
#97347=CARTESIAN_POINT('Ctrl Pts',(20.5849881747801,20.2384495082936,-6.42251797734894));
#97348=CARTESIAN_POINT('Ctrl Pts',(20.5762078322756,20.2540759454207,-6.4214392388114));
#97349=CARTESIAN_POINT('Ctrl Pts',(20.5727798390621,20.2601071587089,-6.42102280835963));
#97350=CARTESIAN_POINT('Ctrl Pts',(20.566111590863,20.2717061873592,-6.42022174937132));
#97351=CARTESIAN_POINT('Ctrl Pts',(20.5628754514984,20.2772762688906,-6.41983697818318));
#97352=CARTESIAN_POINT('Ctrl Pts',(20.5553804521501,20.2900422442813,-6.41895488215932));
#97353=CARTESIAN_POINT('Ctrl Pts',(20.5511042652016,20.2972278807256,-6.41845819292656));
#97354=CARTESIAN_POINT('Ctrl Pts',(20.539570289496,20.3163506654378,-6.41713576716577));
#97355=CARTESIAN_POINT('Ctrl Pts',(20.5322366493738,20.3282417512292,-6.4163128071395));
#97356=CARTESIAN_POINT('Ctrl Pts',(20.4714597550209,20.4246391378215,-6.40963398814145));
#97357=CARTESIAN_POINT('Ctrl Pts',(20.4122054460579,20.5053401891908,-6.40400493477306));
#97358=CARTESIAN_POINT('Ctrl Pts',(20.2361477277666,20.7126004429819,-6.38901948579182));
#97359=CARTESIAN_POINT('Ctrl Pts',(20.1092982871116,20.8295779733223,-6.37998267350489));
#97360=CARTESIAN_POINT('Ctrl Pts',(19.9372872114692,20.9532354276985,-6.36791331017267));
#97361=CARTESIAN_POINT('Ctrl Pts',(19.9042045042924,20.9756261225481,-6.365596850404));
#97362=CARTESIAN_POINT('Ctrl Pts',(19.8640240857614,21.0011937552643,-6.36276398877022));
#97363=CARTESIAN_POINT('Ctrl Pts',(19.8575149910715,21.0052859795811,-6.36230448079656));
#97364=CARTESIAN_POINT('Ctrl Pts',(19.8474096033598,21.0115626229168,-6.36158994396203));
#97365=CARTESIAN_POINT('Ctrl Pts',(19.8438287692874,21.0137719783861,-6.36133652680632));
#97366=CARTESIAN_POINT('Ctrl Pts',(19.8372045120686,21.0178318935702,-6.36086727086378));
#97367=CARTESIAN_POINT('Ctrl Pts',(19.8341629956337,21.019685453459,-6.36065163302646));
#97368=CARTESIAN_POINT('Ctrl Pts',(19.8273126405839,21.0238365220129,-6.36016555465843));
#97369=CARTESIAN_POINT('Ctrl Pts',(19.823501255424,21.0261296921151,-6.35989483812831));
#97370=CARTESIAN_POINT('Ctrl Pts',(19.8137316770894,21.0319658312249,-6.35920028003406));
#97371=CARTESIAN_POINT('Ctrl Pts',(19.8077633105948,21.0354915463709,-6.35877535810323));
#97372=CARTESIAN_POINT('Ctrl Pts',(19.7728187316377,21.0559036334383,-6.35628441180358));
#97373=CARTESIAN_POINT('Ctrl Pts',(19.7434635709076,21.0721278251695,-6.35417977705838));
#97374=CARTESIAN_POINT('Ctrl Pts',(19.6975154986552,21.0961158477308,-6.35088121460067));
#97375=CARTESIAN_POINT('Ctrl Pts',(19.6811848393107,21.1043738984421,-6.34970802781307));
#97376=CARTESIAN_POINT('Ctrl Pts',(19.6425620540246,21.1232798543988,-6.3469347502455));
#97377=CARTESIAN_POINT('Ctrl Pts',(19.6201866552675,21.1337512561645,-6.34532916655376));
#97378=CARTESIAN_POINT('Ctrl Pts',(19.5566233451991,21.1621528575067,-6.34078013147681));
#97379=CARTESIAN_POINT('Ctrl Pts',(19.5150409727976,21.17916703077,-6.33781845401844));
#97380=CARTESIAN_POINT('Ctrl Pts',(19.3704829516139,21.2330125310946,-6.32762833885687));
#97381=CARTESIAN_POINT('Ctrl Pts',(19.2652049043434,21.2631866484315,-6.32039830780838));
#97382=CARTESIAN_POINT('Ctrl Pts',(19.1041214859697,21.2961211436827,-6.30983047334516));
#97383=CARTESIAN_POINT('Ctrl Pts',(19.0497689864349,21.3050417532998,-6.30634427344008));
#97384=CARTESIAN_POINT('Ctrl Pts',(18.9611055016932,21.3160623291872,-6.300790834217));
#97385=CARTESIAN_POINT('Ctrl Pts',(18.9269852360094,21.3194641882862,-6.29868522734318));
#97386=CARTESIAN_POINT('Ctrl Pts',(18.8820200895347,21.3228465439308,-6.29595006980075));
#97387=CARTESIAN_POINT('Ctrl Pts',(18.8712382214932,21.3235746020818,-6.2952972070506));
#97388=CARTESIAN_POINT('Ctrl Pts',(18.853565907974,21.3246320798939,-6.29423187936506));
#97389=CARTESIAN_POINT('Ctrl Pts',(18.8466786887468,21.3250104281578,-6.29381788593897));
#97390=CARTESIAN_POINT('Ctrl Pts',(18.8333408036691,21.3256777761247,-6.2930183901391));
#97391=CARTESIAN_POINT('Ctrl Pts',(18.826890431207,21.3259709362838,-6.29263276163655));
#97392=CARTESIAN_POINT('Ctrl Pts',(18.8119899302177,21.3265798431543,-6.29174425608576));
#97393=CARTESIAN_POINT('Ctrl Pts',(18.803539013247,21.3268744837012,-6.29124204551304));
#97394=CARTESIAN_POINT('Ctrl Pts',(18.780798330885,21.327530944038,-6.28989511001955));
#97395=CARTESIAN_POINT('Ctrl Pts',(18.766506135588,21.3277986883303,-6.28905332875827));
#97396=CARTESIAN_POINT('Ctrl Pts',(18.6350479473451,21.3289296343791,-6.28135182955752));
#97397=CARTESIAN_POINT('Ctrl Pts',(18.5179952710973,21.3202094958374,-6.27481074064599));
#97398=CARTESIAN_POINT('Ctrl Pts',(18.2404054607923,21.2761651782157,-6.25942582748462));
#97399=CARTESIAN_POINT('Ctrl Pts',(18.0821083834066,21.2317839446089,-6.25076841785113));
#97400=CARTESIAN_POINT('Ctrl Pts',(17.9016686478125,21.1577631798093,-6.23955361856694));
#97401=CARTESIAN_POINT('Ctrl Pts',(17.8730712644509,21.1452863897801,-6.23773209066369));
#97402=CARTESIAN_POINT('Ctrl Pts',(17.8382749421488,21.1291805739933,-6.2354486451909));
#97403=CARTESIAN_POINT('Ctrl Pts',(17.8318034794302,21.1261453022322,-6.23502107246662));
#97404=CARTESIAN_POINT('Ctrl Pts',(17.8216539555023,21.121322072134,-6.2343457361428));
#97405=CARTESIAN_POINT('Ctrl Pts',(17.8179654230808,21.1195560975331,-6.23409931402452));
#97406=CARTESIAN_POINT('Ctrl Pts',(17.8110620447559,21.116226315056,-6.23363621153203));
#97407=CARTESIAN_POINT('Ctrl Pts',(17.8078460352514,21.1146650476691,-6.23341968899333));
#97408=CARTESIAN_POINT('Ctrl Pts',(17.8004896490396,21.1110707094039,-6.23292262777543));
#97409=CARTESIAN_POINT('Ctrl Pts',(17.7963519644209,21.1090322538171,-6.23264175658664));
#97410=CARTESIAN_POINT('Ctrl Pts',(17.7855282348213,21.1036558472467,-6.23190369962673));
#97411=CARTESIAN_POINT('Ctrl Pts',(17.7788532122828,21.1002960211633,-6.23144519783144));
#97412=CARTESIAN_POINT('Ctrl Pts',(17.7341725928776,21.0775090411018,-6.22835435280912));
#97413=CARTESIAN_POINT('Ctrl Pts',(17.6967469833069,21.0569730377007,-6.22565941268588));
#97414=CARTESIAN_POINT('Ctrl Pts',(17.6537632117779,21.0316672866917,-6.22246029349298));
#97415=CARTESIAN_POINT('Ctrl Pts',(17.6475745373744,21.0279811775343,-6.2219971112341));
#97416=CARTESIAN_POINT('Ctrl Pts',(17.5067332065525,20.9431162113054,-6.21139884241179));
#97417=CARTESIAN_POINT('Ctrl Pts',(17.381520401944,20.8472189954507,-6.2008255891468));
#97418=CARTESIAN_POINT('Ctrl Pts',(17.199636874156,20.6726489938476,-6.18444646102177));
#97419=CARTESIAN_POINT('Ctrl Pts',(17.1356824216191,20.6024284344092,-6.17842083494831));
#97420=CARTESIAN_POINT('Ctrl Pts',(17.0633767519725,20.5114468083211,-6.17128275661141));
#97421=CARTESIAN_POINT('Ctrl Pts',(17.0503589550626,20.4945485273957,-6.1699827097655));
#97422=CARTESIAN_POINT('Ctrl Pts',(17.0322147355866,20.4702445753607,-6.16814848369047));
#97423=CARTESIAN_POINT('Ctrl Pts',(17.0268770668331,20.4629989144223,-6.1676060504374));
#97424=CARTESIAN_POINT('Ctrl Pts',(17.0177495690939,20.4504418205807,-6.16667346354058));
#97425=CARTESIAN_POINT('Ctrl Pts',(17.0139378254337,20.4451465412564,-6.16628246263704));
#97426=CARTESIAN_POINT('Ctrl Pts',(17.0066870509714,20.4349749098116,-6.16553568459262));
#97427=CARTESIAN_POINT('Ctrl Pts',(17.0032440432675,20.430101481866,-6.16517975662665));
#97428=CARTESIAN_POINT('Ctrl Pts',(16.9943461642458,20.4173932482778,-6.1642564187872));
#97429=CARTESIAN_POINT('Ctrl Pts',(16.9889235640272,20.4095359297471,-6.16369024500889));
#97430=CARTESIAN_POINT('Ctrl Pts',(16.9706219475502,20.3826294503584,-6.16176718777194));
#97431=CARTESIAN_POINT('Ctrl Pts',(16.9579999310821,20.3634068469764,-6.16041999637991));
#97432=CARTESIAN_POINT('Ctrl Pts',(16.8517988254439,20.1957782501648,-6.14888904460162));
#97433=CARTESIAN_POINT('Ctrl Pts',(16.7766910280836,20.0364803167671,-6.13945578366972));
#97434=CARTESIAN_POINT('Ctrl Pts',(16.6950139619086,19.7870198790295,-6.12517347561472));
#97435=CARTESIAN_POINT('Ctrl Pts',(16.6730620310302,19.7027268103163,-6.12040912916544));
#97436=CARTESIAN_POINT('Ctrl Pts',(16.6490998650406,19.5802038588514,-6.1132812613151));
#97437=CARTESIAN_POINT('Ctrl Pts',(16.6428359520119,19.5428924331231,-6.11108386833566));
#97438=CARTESIAN_POINT('Ctrl Pts',(16.6365221765392,19.4979374778731,-6.10838292032738));
#97439=CARTESIAN_POINT('Ctrl Pts',(16.6355092976289,19.4904335417496,-6.10793029751026));
#97440=CARTESIAN_POINT('Ctrl Pts',(16.6339995005659,19.4787767622308,-6.10722420240243));
#97441=CARTESIAN_POINT('Ctrl Pts',(16.6334745843629,19.4746275205329,-6.10697228172458));
#97442=CARTESIAN_POINT('Ctrl Pts',(16.6325251661749,19.4669398822551,-6.10650439881619));
#97443=CARTESIAN_POINT('Ctrl Pts',(16.6320973021977,19.4634019590237,-6.10628862849065));
#97444=CARTESIAN_POINT('Ctrl Pts',(16.6311517266828,19.4554140134578,-6.10580045824318));
#97445=CARTESIAN_POINT('Ctrl Pts',(16.6306392094336,19.4509634439275,-6.10552777130201));
#97446=CARTESIAN_POINT('Ctrl Pts',(16.6291723816807,19.4378600444509,-6.10472293921759));
#97447=CARTESIAN_POINT('Ctrl Pts',(16.6282573256438,19.4292030385308,-6.10418866596148));
#97448=CARTESIAN_POINT('Ctrl Pts',(16.6221408158919,19.3677111227551,-6.10037676936774));
#97449=CARTESIAN_POINT('Ctrl Pts',(16.6188755557929,19.3147070485057,-6.09700299463916));
#97450=CARTESIAN_POINT('Ctrl Pts',(16.6172125017524,19.2452051771546,-6.09251063184672));
#97451=CARTESIAN_POINT('Ctrl Pts',(16.6170107020447,19.2287651447115,-6.09144296094795));
#97452=CARTESIAN_POINT('Ctrl Pts',(16.6169886659552,19.1935499070994,-6.0891472088716));
#97453=CARTESIAN_POINT('Ctrl Pts',(16.6172266779166,19.1747760437117,-6.08791797418893));
#97454=CARTESIAN_POINT('Ctrl Pts',(16.6217705573637,18.9999111347366,-6.07643128804281));
#97455=CARTESIAN_POINT('Ctrl Pts',(16.6430861467256,18.8447196224014,-6.06600971984951));
#97456=CARTESIAN_POINT('Ctrl Pts',(16.6824574159065,18.6886158924888,-6.05574886267654));
#97457=CARTESIAN_POINT('Ctrl Pts',(16.6836494631439,18.6839565419554,-6.05544275861447));
#97458=CARTESIAN_POINT('Ctrl Pts',(16.7007616129654,18.6180070985914,-6.05111241008373));
#97459=CARTESIAN_POINT('Ctrl Pts',(16.7194091022808,18.5574529387656,-6.04716616922773));
#97460=CARTESIAN_POINT('Ctrl Pts',(16.7422893639867,18.4935052270817,-6.04302901175127));
#97461=CARTESIAN_POINT('Ctrl Pts',(16.7438474130825,18.4891948409118,-6.04275028930809));
#97462=CARTESIAN_POINT('Ctrl Pts',(16.7454194503114,18.4848895418737,-6.04247203357104));
#97463=CARTESIAN_POINT('Origin',(18.734,19.211,0.));
#97464=CARTESIAN_POINT('',(16.745419381199,18.4848897311503,-5.24452701096004));
#97465=CARTESIAN_POINT('',(16.7454194503191,18.4848895418526,-5.46434828430915));
#97466=CARTESIAN_POINT('',(16.7454194503191,18.4848895418526,0.));
#97467=CARTESIAN_POINT('',(16.6170006442152,19.2093484532524,-5.51218499391188));
#97468=CARTESIAN_POINT('Ctrl Pts',(16.7454194503191,18.4848895418527,-5.46434828430915));
#97469=CARTESIAN_POINT('Ctrl Pts',(16.7446923999496,18.4868806965141,-5.4644758422322));
#97470=CARTESIAN_POINT('Ctrl Pts',(16.7439683437551,18.4888729333669,-5.46460357631697));
#97471=CARTESIAN_POINT('Ctrl Pts',(16.7420339915519,18.4942202967959,-5.46494672233998));
#97472=CARTESIAN_POINT('Ctrl Pts',(16.7408292055697,18.4975773302596,-5.46516246031084));
#97473=CARTESIAN_POINT('Ctrl Pts',(16.7382405876864,18.5048480337378,-5.46563039949849));
#97474=CARTESIAN_POINT('Ctrl Pts',(16.7368598003935,18.5087626799101,-5.46588277144038));
#97475=CARTESIAN_POINT('Ctrl Pts',(16.7330402093437,18.5196939195587,-5.46658863297378));
#97476=CARTESIAN_POINT('Ctrl Pts',(16.7306268379231,18.5267192459324,-5.46704358502534));
#97477=CARTESIAN_POINT('Ctrl Pts',(16.7169221932686,18.5673074602492,-5.46967895501753));
#97478=CARTESIAN_POINT('Ctrl Pts',(16.70643819295,18.6011346529457,-5.47190251098958));
#97479=CARTESIAN_POINT('Ctrl Pts',(16.6756286877856,18.7101405100038,-5.47911945319092));
#97480=CARTESIAN_POINT('Ctrl Pts',(16.6586012281405,18.7861812344539,-5.48422947167187));
#97481=CARTESIAN_POINT('Ctrl Pts',(16.6267248929344,18.977447016726,-5.497026588454));
#97482=CARTESIAN_POINT('Ctrl Pts',(16.617091182629,19.0932937524003,-5.50471798017525));
#97483=CARTESIAN_POINT('Ctrl Pts',(16.6170006442152,19.2093484532524,-5.51218499391188));
#97484=CARTESIAN_POINT('Ctrl Pts',(16.6170006421798,19.2093510643075,-5.51218516190835));
#97485=CARTESIAN_POINT('Ctrl Pts',(16.6169350228221,19.2935970047459,-5.517605582707));
#97486=CARTESIAN_POINT('Ctrl Pts',(16.6218981977752,19.3777818118907,-5.52290047725799));
#97487=CARTESIAN_POINT('Ctrl Pts',(16.6330988038497,19.471789986764,-5.52867286592509));
#97488=CARTESIAN_POINT('Ctrl Pts',(16.6344059037781,19.4821123205625,-5.52930484381016));
#97489=CARTESIAN_POINT('Ctrl Pts',(16.636738347915,19.4995022617998,-5.53036650859551));
#97490=CARTESIAN_POINT('Ctrl Pts',(16.6377234400716,19.5065749966085,-5.53079745786133));
#97491=CARTESIAN_POINT('Ctrl Pts',(16.6396009364873,19.5195732790937,-5.53158794109212));
#97492=CARTESIAN_POINT('Ctrl Pts',(16.6404827460144,19.5255002610929,-5.53194780640628));
#97493=CARTESIAN_POINT('Ctrl Pts',(16.6423536689177,19.5377188184431,-5.53268850407761));
#97494=CARTESIAN_POINT('Ctrl Pts',(16.6433460333441,19.5440098402922,-5.53306922932213));
#97495=CARTESIAN_POINT('Ctrl Pts',(16.6456303020622,19.5580780255571,-5.53391922565105));
#97496=CARTESIAN_POINT('Ctrl Pts',(16.6469372945572,19.5658526697254,-5.53438801268315));
#97497=CARTESIAN_POINT('Ctrl Pts',(16.6503587999105,19.5855324378407,-5.53557231933836));
#97498=CARTESIAN_POINT('Ctrl Pts',(16.6525319505521,19.5974271806305,-5.53628597239032));
#97499=CARTESIAN_POINT('Ctrl Pts',(16.6655166081195,19.6652087964251,-5.54034126659226));
#97500=CARTESIAN_POINT('Ctrl Pts',(16.6784773190028,19.720663137167,-5.5436137078366));
#97501=CARTESIAN_POINT('Ctrl Pts',(16.7044778513509,19.8146348024952,-5.54912152047655));
#97502=CARTESIAN_POINT('Ctrl Pts',(16.7164193736241,19.8534202410136,-5.55138376998296));
#97503=CARTESIAN_POINT('Ctrl Pts',(16.7740763462376,20.0231741252782,-5.56128903855644));
#97504=CARTESIAN_POINT('Ctrl Pts',(16.8314807496511,20.1498001938405,-5.56866564273553));
#97505=CARTESIAN_POINT('Ctrl Pts',(16.9272998012879,20.3156803760131,-5.5792670548473));
#97506=CARTESIAN_POINT('Ctrl Pts',(16.955449295854,20.3604524660741,-5.58223563216153));
#97507=CARTESIAN_POINT('Ctrl Pts',(17.0008241867492,20.4269584435849,-5.58688419654007));
#97508=CARTESIAN_POINT('Ctrl Pts',(17.0168505965829,20.4494874230843,-5.58850295395942));
#97509=CARTESIAN_POINT('Ctrl Pts',(17.0374075367327,20.4772188974816,-5.59056000568632));
#97510=CARTESIAN_POINT('Ctrl Pts',(17.0415292359698,20.4827228442926,-5.59097151644611));
#97511=CARTESIAN_POINT('Ctrl Pts',(17.0481085688684,20.4914199772946,-5.5916271016444));
#97512=CARTESIAN_POINT('Ctrl Pts',(17.0505486724653,20.4946264499519,-5.59186996237869));
#97513=CARTESIAN_POINT('Ctrl Pts',(17.0551780844881,20.5006739279624,-5.59233023868622));
#97514=CARTESIAN_POINT('Ctrl Pts',(17.0573654641445,20.5035163429982,-5.59254751940847));
#97515=CARTESIAN_POINT('Ctrl Pts',(17.0623961945627,20.5100193232251,-5.59304677427222));
#97516=CARTESIAN_POINT('Ctrl Pts',(17.0652443490526,20.5136761151391,-5.59332908639859));
#97517=CARTESIAN_POINT('Ctrl Pts',(17.0728655611403,20.5233951038866,-5.59408353521667));
#97518=CARTESIAN_POINT('Ctrl Pts',(17.0776597391594,20.5294405442933,-5.59455711801425));
#97519=CARTESIAN_POINT('Ctrl Pts',(17.1122279307319,20.5725447872489,-5.59796386322302));
#97520=CARTESIAN_POINT('Ctrl Pts',(17.1432073900363,20.608614740661,-5.60097459101504));
#97521=CARTESIAN_POINT('Ctrl Pts',(17.1951783807622,20.6651573822001,-5.6059183148775));
#97522=CARTESIAN_POINT('Ctrl Pts',(17.2154292583923,20.686292669097,-5.60782052074561));
#97523=CARTESIAN_POINT('Ctrl Pts',(17.2868157387307,20.7577692559931,-5.61442594194357));
#97524=CARTESIAN_POINT('Ctrl Pts',(17.3400677892033,20.8059263580313,-5.61918105526391));
#97525=CARTESIAN_POINT('Ctrl Pts',(17.4767036864319,20.9174100614128,-5.63082310362648));
#97526=CARTESIAN_POINT('Ctrl Pts',(17.5625427734562,20.9774431558819,-5.63766787015467));
#97527=CARTESIAN_POINT('Ctrl Pts',(17.6871080699928,21.0514698403135,-5.64685779627215));
#97528=CARTESIAN_POINT('Ctrl Pts',(17.7223220099948,21.0710591191976,-5.6493812006332));
#97529=CARTESIAN_POINT('Ctrl Pts',(17.7742766688073,21.0980488708036,-5.65299758058682));
#97530=CARTESIAN_POINT('Ctrl Pts',(17.7905864472094,21.1062554483016,-5.65411804418506));
#97531=CARTESIAN_POINT('Ctrl Pts',(17.8200118227736,21.120587405612,-5.65611352202763));
#97532=CARTESIAN_POINT('Ctrl Pts',(17.83308777644,21.1267911236725,-5.65699120926473));
#97533=CARTESIAN_POINT('Ctrl Pts',(17.8531817375395,21.1360732154926,-5.65832641127633));
#97534=CARTESIAN_POINT('Ctrl Pts',(17.8601543557683,21.1392482954628,-5.65878725732571));
#97535=CARTESIAN_POINT('Ctrl Pts',(17.872950307635,21.1449914503523,-5.65962853019147));
#97536=CARTESIAN_POINT('Ctrl Pts',(17.878768256399,21.1475712403278,-5.66000935620905));
#97537=CARTESIAN_POINT('Ctrl Pts',(17.8913115781374,21.1530656392479,-5.66082684493576));
#97538=CARTESIAN_POINT('Ctrl Pts',(17.8980406479681,21.1559716417756,-5.6612632095029));
#97539=CARTESIAN_POINT('Ctrl Pts',(17.9162253257146,21.1637130330821,-5.6624366333298));
#97540=CARTESIAN_POINT('Ctrl Pts',(17.9277087764944,21.1684825874829,-5.66317145057699));
#97541=CARTESIAN_POINT('Ctrl Pts',(17.9825479372701,21.1906951074065,-5.6666520442154));
#97542=CARTESIAN_POINT('Ctrl Pts',(18.0264332470636,21.206801264651,-5.66935264452889));
#97543=CARTESIAN_POINT('Ctrl Pts',(18.2543902931222,21.2819971200523,-5.68301461480048));
#97544=CARTESIAN_POINT('Ctrl Pts',(18.4453739919648,21.3171209258884,-5.69315886758305));
#97545=CARTESIAN_POINT('Ctrl Pts',(18.6897804587139,21.3281613038901,-5.706714952772));
#97546=CARTESIAN_POINT('Ctrl Pts',(18.7411570699376,21.3286107812708,-5.70960274343206));
#97547=CARTESIAN_POINT('Ctrl Pts',(18.8196003149383,21.3264424644324,-5.71413655144819));
#97548=CARTESIAN_POINT('Ctrl Pts',(18.8466868366006,21.3251725933766,-5.71572488545301));
#97549=CARTESIAN_POINT('Ctrl Pts',(18.880557488857,21.3229319552709,-5.71774786777438));
#97550=CARTESIAN_POINT('Ctrl Pts',(18.8873726251609,21.3224479667229,-5.71815678419441));
#97551=CARTESIAN_POINT('Ctrl Pts',(18.8981932883466,21.3216268550834,-5.71880917781701));
#97552=CARTESIAN_POINT('Ctrl Pts',(18.902200471189,21.3213112941483,-5.71905146144865));
#97553=CARTESIAN_POINT('Ctrl Pts',(18.9097837904224,21.3206923803924,-5.71951130382944));
#97554=CARTESIAN_POINT('Ctrl Pts',(18.9133600632854,21.3203913453468,-5.71972873153826));
#97555=CARTESIAN_POINT('Ctrl Pts',(18.9215704941605,21.3196791966192,-5.72022919158013));
#97556=CARTESIAN_POINT('Ctrl Pts',(18.9262040716622,21.319261899864,-5.72051256765587));
#97557=CARTESIAN_POINT('Ctrl Pts',(18.9385770418966,21.3181064703368,-5.7212717060231));
#97558=CARTESIAN_POINT('Ctrl Pts',(18.9463137228883,21.3173409795743,-5.72174894236395));
#97559=CARTESIAN_POINT('Ctrl Pts',(19.0026924205808,21.3114489320931,-5.72524443535702));
#97560=CARTESIAN_POINT('Ctrl Pts',(19.0511441512915,21.304680992576,-5.7283447803929));
#97561=CARTESIAN_POINT('Ctrl Pts',(19.2504330645577,21.269767563705,-5.74138160112831));
#97562=CARTESIAN_POINT('Ctrl Pts',(19.3982263174172,21.2269446504282,-5.7516915156213));
#97563=CARTESIAN_POINT('Ctrl Pts',(19.6311631791648,21.1310225334437,-5.76808693086142));
#97564=CARTESIAN_POINT('Ctrl Pts',(19.7195108098392,21.0872093152235,-5.77435330579763));
#97565=CARTESIAN_POINT('Ctrl Pts',(19.8232681037661,21.0263945574511,-5.78174347041408));
#97566=CARTESIAN_POINT('Ctrl Pts',(19.841868960817,21.0151033291436,-5.78307001482165));
#97567=CARTESIAN_POINT('Ctrl Pts',(19.8679739231567,20.9987008781262,-5.78493475864143));
#97568=CARTESIAN_POINT('Ctrl Pts',(19.8756238356116,20.9938253728339,-5.78548159014019));
#97569=CARTESIAN_POINT('Ctrl Pts',(19.8887327029067,20.9853517479328,-5.78641937018984));
#97570=CARTESIAN_POINT('Ctrl Pts',(19.894206715364,20.9817772642732,-5.78681119100015));
#97571=CARTESIAN_POINT('Ctrl Pts',(19.9046328341177,20.9748999964293,-5.78755793698989));
#97572=CARTESIAN_POINT('Ctrl Pts',(19.9095877321843,20.9716015775211,-5.78791302068994));
#97573=CARTESIAN_POINT('Ctrl Pts',(19.9223859275535,20.9630038485013,-5.78883074298802));
#97574=CARTESIAN_POINT('Ctrl Pts',(19.930207767615,20.9576727166509,-5.78939217576493));
#97575=CARTESIAN_POINT('Ctrl Pts',(19.9565036081274,20.9394907711702,-5.7912817371614));
#97576=CARTESIAN_POINT('Ctrl Pts',(19.9748087767351,20.9263976374844,-5.79260063350919));
#97577=CARTESIAN_POINT('Ctrl Pts',(20.138770260746,20.8051228485415,-5.80445696454059));
#97578=CARTESIAN_POINT('Ctrl Pts',(20.270161527352,20.6789309431317,-5.81418241168746));
#97579=CARTESIAN_POINT('Ctrl Pts',(20.4358105302999,20.4729048502185,-5.82858160045585));
#97580=CARTESIAN_POINT('Ctrl Pts',(20.4839171255178,20.405299303186,-5.83313262327671));
#97581=CARTESIAN_POINT('Ctrl Pts',(20.5474539765932,20.3038977391938,-5.83997218089297));
#97582=CARTESIAN_POINT('Ctrl Pts',(20.5661595705515,20.2722406573064,-5.84210956695578));
#97583=CARTESIAN_POINT('Ctrl Pts',(20.5876810783615,20.2335516440555,-5.84474398796897));
#97584=CARTESIAN_POINT('Ctrl Pts',(20.5912969814934,20.2269691549152,-5.84519296543809));
#97585=CARTESIAN_POINT('Ctrl Pts',(20.5968654300036,20.2167031220242,-5.84589458873561));
#97586=CARTESIAN_POINT('Ctrl Pts',(20.5988422903456,20.2130327396858,-5.84614571435808));
#97587=CARTESIAN_POINT('Ctrl Pts',(20.6024894826581,20.2062129230567,-5.84661287935017));
#97588=CARTESIAN_POINT('Ctrl Pts',(20.6041627056437,20.2030651001051,-5.8468287316553));
#97589=CARTESIAN_POINT('Ctrl Pts',(20.6079289510642,20.1959363000461,-5.84731806575701));
#97590=CARTESIAN_POINT('Ctrl Pts',(20.6100172313672,20.1919528915984,-5.8475918406436));
#97591=CARTESIAN_POINT('Ctrl Pts',(20.6161479708735,20.1801672878839,-5.84840280394313));
#97592=CARTESIAN_POINT('Ctrl Pts',(20.6201545053846,20.1723466553952,-5.84894216823161));
#97593=CARTESIAN_POINT('Ctrl Pts',(20.6489204465247,20.1153243465001,-5.85288248004627));
#97594=CARTESIAN_POINT('Ctrl Pts',(20.6717978310808,20.0652021296956,-5.85638687731439));
#97595=CARTESIAN_POINT('Ctrl Pts',(20.7564685845423,19.8587359217368,-5.87082506437484));
#97596=CARTESIAN_POINT('Ctrl Pts',(20.8014990086526,19.6961767047059,-5.88214040023727));
#97597=CARTESIAN_POINT('Ctrl Pts',(20.838952647047,19.4504510447495,-5.89816375150085));
#97598=CARTESIAN_POINT('Ctrl Pts',(20.8465329400232,19.370278524744,-5.90323925098005));
#97599=CARTESIAN_POINT('Ctrl Pts',(20.8502581499253,19.2703449460948,-5.90937017786263));
#97600=CARTESIAN_POINT('Ctrl Pts',(20.8507155673185,19.2508199314504,-5.91055901552437));
#97601=CARTESIAN_POINT('Ctrl Pts',(20.8509860039086,19.2226058436378,-5.9122643639514));
#97602=CARTESIAN_POINT('Ctrl Pts',(20.8510158033641,19.2139203031908,-5.91278763002537));
#97603=CARTESIAN_POINT('Ctrl Pts',(20.8509745295113,19.1987646703921,-5.91369776713135));
#97604=CARTESIAN_POINT('Ctrl Pts',(20.850927248219,19.1922946777547,-5.91408537814049));
#97605=CARTESIAN_POINT('Ctrl Pts',(20.8507784687399,19.1797845197975,-5.91483308798317));
#97606=CARTESIAN_POINT('Ctrl Pts',(20.8506807770335,19.1737443799408,-5.91519330221259));
#97607=CARTESIAN_POINT('Ctrl Pts',(20.8503871358699,19.1593892832168,-5.91604754545429));
#97608=CARTESIAN_POINT('Ctrl Pts',(20.8501680357624,19.1510748601889,-5.91654084616701));
#97609=CARTESIAN_POINT('Ctrl Pts',(20.8492155476901,19.1215405081676,-5.91828807443887));
#97610=CARTESIAN_POINT('Ctrl Pts',(20.8482119193869,19.1003301215115,-5.91953355375152));
#97611=CARTESIAN_POINT('Ctrl Pts',(20.8348468506118,18.8861753481645,-5.93202434393746));
#97612=CARTESIAN_POINT('Ctrl Pts',(20.7964311119478,18.6957800196862,-5.94232524204041));
#97613=CARTESIAN_POINT('Ctrl Pts',(20.7079197406423,18.4422456443887,-5.95699095690298));
#97614=CARTESIAN_POINT('Ctrl Pts',(20.6793748141262,18.3726340348035,-5.96114001020319));
#97615=CARTESIAN_POINT('Ctrl Pts',(20.6323507349037,18.2733673017251,-5.96743216391842));
#97616=CARTESIAN_POINT('Ctrl Pts',(20.6167445704538,18.2424117700734,-5.96945054876323));
#97617=CARTESIAN_POINT('Ctrl Pts',(20.5969027965435,18.2053476455521,-5.97195291795997));
#97618=CARTESIAN_POINT('Ctrl Pts',(20.5933850240021,18.1988583022872,-5.97239429007523));
#97619=CARTESIAN_POINT('Ctrl Pts',(20.5878410500989,18.1887576082805,-5.97308657874437));
#97620=CARTESIAN_POINT('Ctrl Pts',(20.5858380291481,18.1851335079134,-5.97333603970697));
#97621=CARTESIAN_POINT('Ctrl Pts',(20.58208935195,18.1783977158511,-5.97380172914152));
#97622=CARTESIAN_POINT('Ctrl Pts',(20.5803464574785,18.1752845524217,-5.97401778077037));
#97623=CARTESIAN_POINT('Ctrl Pts',(20.5763697942239,18.168223361461,-5.97450967737042));
#97624=CARTESIAN_POINT('Ctrl Pts',(20.5741312109305,18.1642781161047,-5.97478582866334));
#97625=CARTESIAN_POINT('Ctrl Pts',(20.5682967111223,18.1540720438649,-5.97550357216521));
#97626=CARTESIAN_POINT('Ctrl Pts',(20.5646814488057,18.1478224238316,-5.97594636771421));
#97627=CARTESIAN_POINT('Ctrl Pts',(20.5417965212058,18.1087245957527,-5.97873661985179));
#97628=CARTESIAN_POINT('Ctrl Pts',(20.521676651128,18.0763850411015,-5.98113391110635));
#97629=CARTESIAN_POINT('Ctrl Pts',(20.4932674544053,18.0333545240416,-5.98442854375312));
#97630=CARTESIAN_POINT('Ctrl Pts',(20.4857305261716,18.0221724293492,-5.98529459231634));
#97631=CARTESIAN_POINT('Ctrl Pts',(20.4776250015664,18.0103911879699,-5.98621700962352));
#97632=CARTESIAN_POINT('Ctrl Pts',(20.4771621814781,18.009719318946,-5.98626964852478));
#97633=CARTESIAN_POINT('Ctrl Pts',(20.463734896018,17.9902512277851,-5.98779591518946));
#97634=CARTESIAN_POINT('Ctrl Pts',(20.4504678796014,17.9716661703838,-5.98927998968137));
#97635=CARTESIAN_POINT('Ctrl Pts',(20.4097693768218,17.9165611363241,-5.99375469302987));
#97636=CARTESIAN_POINT('Ctrl Pts',(20.3814543577333,17.8807109619743,-5.9967659934363));
#97637=CARTESIAN_POINT('Ctrl Pts',(20.2814846348372,17.7622287298823,-6.00700641737681));
#97638=CARTESIAN_POINT('Ctrl Pts',(20.2045912957222,17.6842349245166,-6.01423699864965));
#97639=CARTESIAN_POINT('Ctrl Pts',(20.080434069921,17.576424703056,-6.02480598858788));
#97640=CARTESIAN_POINT('Ctrl Pts',(20.0374614790086,17.5419553336429,-6.02829278990761));
#97641=CARTESIAN_POINT('Ctrl Pts',(19.9656280397148,17.488804606175,-6.03384707504526));
#97642=CARTESIAN_POINT('Ctrl Pts',(19.9375730048731,17.4690824242569,-6.03595294098667));
#97643=CARTESIAN_POINT('Ctrl Pts',(19.9000608485796,17.4440512515222,-6.03868838078686));
#97644=CARTESIAN_POINT('Ctrl Pts',(19.8910258522233,17.4381218410713,-6.03934127274135));
#97645=CARTESIAN_POINT('Ctrl Pts',(19.8761502341641,17.4285215514451,-6.04040663591698));
#97646=CARTESIAN_POINT('Ctrl Pts',(19.8703364549321,17.4248096294325,-6.04082063582467));
#97647=CARTESIAN_POINT('Ctrl Pts',(19.8590454247469,17.4176780869468,-6.04162013573756));
#97648=CARTESIAN_POINT('Ctrl Pts',(19.8535704733016,17.4142549851697,-6.04200576191569));
#97649=CARTESIAN_POINT('Ctrl Pts',(19.8408898465981,17.4064071469845,-6.04289425009978));
#97650=CARTESIAN_POINT('Ctrl Pts',(19.8336731207864,17.4020004067881,-6.04339644571447));
#97651=CARTESIAN_POINT('Ctrl Pts',(19.8141869496983,17.3902612902263,-6.04474331443113));
#97652=CARTESIAN_POINT('Ctrl Pts',(19.8018691952349,17.3830096574772,-6.04558504433651));
#97653=CARTESIAN_POINT('Ctrl Pts',(19.6879717255663,17.3175008274633,-6.05328243071551));
#97654=CARTESIAN_POINT('Ctrl Pts',(19.5817897989261,17.2676372147659,-6.0598198657114));
#97655=CARTESIAN_POINT('Ctrl Pts',(19.3186488425677,17.1697625834431,-6.0751882390939));
#97656=CARTESIAN_POINT('Ctrl Pts',(19.1592049339455,17.1306988251208,-6.08383348734822));
#97657=CARTESIAN_POINT('Ctrl Pts',(18.965647465654,17.1064765451146,-6.09504684896966));
#97658=CARTESIAN_POINT('Ctrl Pts',(18.9343371089752,17.10326559435,-6.09688396807863));
#97659=CARTESIAN_POINT('Ctrl Pts',(18.895824122615,17.1001818348265,-6.09918477932821));
#97660=CARTESIAN_POINT('Ctrl Pts',(18.8886767441527,17.0996460565407,-6.09961350528181));
#97661=CARTESIAN_POINT('Ctrl Pts',(18.877443026798,17.0988613072369,-6.10029025902922));
#97662=CARTESIAN_POINT('Ctrl Pts',(18.8733583749534,17.0985878711574,-6.10053693595945));
#97663=CARTESIAN_POINT('Ctrl Pts',(18.8657059629365,17.0980978926574,-6.10100024967099));
#97664=CARTESIAN_POINT('Ctrl Pts',(18.8621384387727,17.0978785373947,-6.10121672700388));
#97665=CARTESIAN_POINT('Ctrl Pts',(18.8539725124614,17.0973971966867,-6.10171332906332));
#97666=CARTESIAN_POINT('Ctrl Pts',(18.8493738138443,17.097141183505,-6.10199378399335));
#97667=CARTESIAN_POINT('Ctrl Pts',(18.8351628252793,17.0963965577087,-6.10286281490277));
#97668=CARTESIAN_POINT('Ctrl Pts',(18.825548167811,17.0959584967884,-6.10345411067238));
#97669=CARTESIAN_POINT('Ctrl Pts',(18.7294013803014,17.0922346823894,-6.10939821466919));
#97670=CARTESIAN_POINT('Ctrl Pts',(18.642757057258,17.094196071647,-6.11500401293072));
#97671=CARTESIAN_POINT('Ctrl Pts',(18.4300124818302,17.1120979616639,-6.12902164966085));
#97672=CARTESIAN_POINT('Ctrl Pts',(18.3047409103902,17.1340940355241,-6.13748303995429));
#97673=CARTESIAN_POINT('Ctrl Pts',(18.0889892910458,17.1923444314256,-6.1519472826074));
#97674=CARTESIAN_POINT('Ctrl Pts',(17.9976065264711,17.2238567469128,-6.15804196483319));
#97675=CARTESIAN_POINT('Ctrl Pts',(17.8952172280175,17.2672031287852,-6.16482089800075));
#97676=CARTESIAN_POINT('Ctrl Pts',(17.8818109407093,17.2730431792278,-6.16570765742976));
#97677=CARTESIAN_POINT('Ctrl Pts',(17.8614116592003,17.2821821395861,-6.16705592614929));
#97678=CARTESIAN_POINT('Ctrl Pts',(17.854374640313,17.2853811435752,-6.16752083979656));
#97679=CARTESIAN_POINT('Ctrl Pts',(17.8415803469013,17.2912821545212,-6.16836582331309));
#97680=CARTESIAN_POINT('Ctrl Pts',(17.8358174497876,17.2939716873904,-6.16874631704546));
#97681=CARTESIAN_POINT('Ctrl Pts',(17.8233758159176,17.299846592923,-6.16956757408814));
#97682=CARTESIAN_POINT('Ctrl Pts',(17.8167014675494,17.3030411025095,-6.17000801513585));
#97683=CARTESIAN_POINT('Ctrl Pts',(17.7985847191415,17.3118292690789,-6.1712032885805));
#97684=CARTESIAN_POINT('Ctrl Pts',(17.7871757129363,17.317491353878,-6.17195573327384));
#97685=CARTESIAN_POINT('Ctrl Pts',(17.7311353669005,17.3459363325564,-6.1756512359713));
#97686=CARTESIAN_POINT('Ctrl Pts',(17.6872695017149,17.3701969683445,-6.17854192764237));
#97687=CARTESIAN_POINT('Ctrl Pts',(17.495479817139,17.4853439641728,-6.19124129427989));
#97688=CARTESIAN_POINT('Ctrl Pts',(17.3582178149021,17.5926538521584,-6.20043477883872));
#97689=CARTESIAN_POINT('Ctrl Pts',(17.1912971852306,17.7599007014551,-6.21342102395247));
#97690=CARTESIAN_POINT('Ctrl Pts',(17.1489970496455,17.8062275459842,-6.21691351441275));
#97691=CARTESIAN_POINT('Ctrl Pts',(17.0889997154134,17.8781010873936,-6.2222987706409));
#97692=CARTESIAN_POINT('Ctrl Pts',(17.069704840534,17.9022728158016,-6.22410479523322));
#97693=CARTESIAN_POINT('Ctrl Pts',(17.0466234996822,17.9325242042836,-6.22637096767601));
#97694=CARTESIAN_POINT('Ctrl Pts',(17.0423282334413,17.9382131187843,-6.22679738284875));
#97695=CARTESIAN_POINT('Ctrl Pts',(17.0356167567508,17.9471961988009,-6.22747129638371));
#97696=CARTESIAN_POINT('Ctrl Pts',(17.0331811649679,17.9504759111282,-6.22771746265424));
#97697=CARTESIAN_POINT('Ctrl Pts',(17.0286315569541,17.9566395018317,-6.22818035429558));
#97698=CARTESIAN_POINT('Ctrl Pts',(17.0265153490006,17.9595216934266,-6.22839692345473));
#97699=CARTESIAN_POINT('Ctrl Pts',(17.0216819493963,17.96613967337,-6.22889445122355));
#97700=CARTESIAN_POINT('Ctrl Pts',(17.0189696844426,17.9698789925934,-6.22917574468107));
#97701=CARTESIAN_POINT('Ctrl Pts',(17.0106032963251,17.9814932751574,-6.23004991216945));
#97702=CARTESIAN_POINT('Ctrl Pts',(17.0049911059434,17.9893980923637,-6.23064555170152));
#97703=CARTESIAN_POINT('Ctrl Pts',(16.942141687169,18.079222742175,-6.23741892762844));
#97704=CARTESIAN_POINT('Ctrl Pts',(16.8907261962258,18.1650492762821,-6.2439318518382));
#97705=CARTESIAN_POINT('Ctrl Pts',(16.8076114310492,18.3290878318613,-6.25604811786295));
#97706=CARTESIAN_POINT('Ctrl Pts',(16.774176965914,18.4061320945035,-6.26161627532157));
#97707=CARTESIAN_POINT('Ctrl Pts',(16.7454195730112,18.484889205839,-6.26710634208694));
#97708=CARTESIAN_POINT('',(16.617000284924,19.2120983478179,-5.28730622481232));
#97709=CARTESIAN_POINT('Ctrl Pts',(16.7454194503114,18.4848895418737,-6.04247203357104));
#97710=CARTESIAN_POINT('Ctrl Pts',(16.7481387459572,18.4774422749056,-6.0419907093376));
#97711=CARTESIAN_POINT('Ctrl Pts',(16.750899896563,18.4700102295166,-6.04151078181624));
#97712=CARTESIAN_POINT('Ctrl Pts',(16.75653554949,18.4550981841722,-6.04054860862168));
#97713=CARTESIAN_POINT('Ctrl Pts',(16.7594108865832,18.4476186771125,-6.04006640307945));
#97714=CARTESIAN_POINT('Ctrl Pts',(16.7646516664199,18.4342137728658,-6.03920284167889));
#97715=CARTESIAN_POINT('Ctrl Pts',(16.7670015473001,18.4282824327406,-6.0388209688949));
#97716=CARTESIAN_POINT('Ctrl Pts',(16.772057849224,18.4156863902265,-6.03801046316236));
#97717=CARTESIAN_POINT('Ctrl Pts',(16.7747715031624,18.4090246637072,-6.03758207989412));
#97718=CARTESIAN_POINT('Ctrl Pts',(16.7821570484165,18.3911551801844,-6.0364336365191));
#97719=CARTESIAN_POINT('Ctrl Pts',(16.7868915427081,18.3799734655095,-6.03571570389965));
#97720=CARTESIAN_POINT('Ctrl Pts',(16.8108499540655,18.3247185221913,-6.03217069704112));
#97721=CARTESIAN_POINT('Ctrl Pts',(16.8314761708487,18.2812664059025,-6.02939191354512));
#97722=CARTESIAN_POINT('Ctrl Pts',(16.9305768783373,18.089634205546,-6.01711723884615));
#97723=CARTESIAN_POINT('Ctrl Pts',(17.0250011761165,17.9503966729864,-6.00819925148187));
#97724=CARTESIAN_POINT('Ctrl Pts',(17.1995518208954,17.7491852038798,-5.99361572799738));
#97725=CARTESIAN_POINT('Ctrl Pts',(17.2693672178715,17.6792430339765,-5.98812308154839));
#97726=CARTESIAN_POINT('Ctrl Pts',(17.3511068478608,17.608068459226,-5.98170194445832));
#97727=CARTESIAN_POINT('Ctrl Pts',(17.3584620215311,17.6017522700469,-5.98112420622296));
#97728=CARTESIAN_POINT('Ctrl Pts',(17.3693853989644,17.5925015196791,-5.98026582349408));
#97729=CARTESIAN_POINT('Ctrl Pts',(17.3729203611462,17.5895276579816,-5.97998798233413));
#97730=CARTESIAN_POINT('Ctrl Pts',(17.3792087466636,17.5842724734305,-5.97949356993484));
#97731=CARTESIAN_POINT('Ctrl Pts',(17.3819582460405,17.5819865313151,-5.97927734067681));
#97732=CARTESIAN_POINT('Ctrl Pts',(17.3878614400866,17.5771038387136,-5.97881295987964));
#97733=CARTESIAN_POINT('Ctrl Pts',(17.3910168158717,17.5745092866599,-5.97856466208833));
#97734=CARTESIAN_POINT('Ctrl Pts',(17.3996985526611,17.5674126255078,-5.97788132970049));
#97735=CARTESIAN_POINT('Ctrl Pts',(17.4052401142961,17.5629293180289,-5.97744497757514));
#97736=CARTESIAN_POINT('Ctrl Pts',(17.4349421976595,17.5391465285037,-5.97510571392364));
#97737=CARTESIAN_POINT('Ctrl Pts',(17.4594994156479,17.520351239543,-5.97317002985472));
#97738=CARTESIAN_POINT('Ctrl Pts',(17.5350662199068,17.4650969832626,-5.96723066083318));
#97739=CARTESIAN_POINT('Ctrl Pts',(17.5872900516001,17.4303611403505,-5.96314954571131));
#97740=CARTESIAN_POINT('Ctrl Pts',(17.7561737873169,17.3285443011583,-5.95019052796835));
#97741=CARTESIAN_POINT('Ctrl Pts',(17.8777423238762,17.2702239827259,-5.94122487589165));
#97742=CARTESIAN_POINT('Ctrl Pts',(18.0423575416279,17.2097535817557,-5.92993142637269));
#97743=CARTESIAN_POINT('Ctrl Pts',(18.0810894552583,17.1967843569459,-5.92732948001112));
#97744=CARTESIAN_POINT('Ctrl Pts',(18.1665837488862,17.1708825180933,-5.92171050301941));
#97745=CARTESIAN_POINT('Ctrl Pts',(18.2134653624909,17.1584199558639,-5.91870889039176));
#97746=CARTESIAN_POINT('Ctrl Pts',(18.2730119751691,17.1447624420808,-5.91499302062857));
#97747=CARTESIAN_POINT('Ctrl Pts',(18.285312165364,17.1420565878713,-5.91423055232542));
#97748=CARTESIAN_POINT('Ctrl Pts',(18.3048443022585,17.1379421974862,-5.9130276817962));
#97749=CARTESIAN_POINT('Ctrl Pts',(18.3120605692159,17.1364614044675,-5.91258497417978));
#97750=CARTESIAN_POINT('Ctrl Pts',(18.3255226960721,17.1337720971466,-5.91176220923687));
#97751=CARTESIAN_POINT('Ctrl Pts',(18.3317665392016,17.1325540149916,-5.91138185021932));
#97752=CARTESIAN_POINT('Ctrl Pts',(18.3456487636471,17.1299106960005,-5.91053890480252));
#97753=CARTESIAN_POINT('Ctrl Pts',(18.3532897163211,17.1284993262035,-5.91007676503983));
#97754=CARTESIAN_POINT('Ctrl Pts',(18.3755207663398,17.1245194462317,-5.90873738689269));
#97755=CARTESIAN_POINT('Ctrl Pts',(18.3901304558915,17.1220619407117,-5.90786367991764));
#97756=CARTESIAN_POINT('Ctrl Pts',(18.5067614704049,17.1037001210185,-5.90093807258743));
#97757=CARTESIAN_POINT('Ctrl Pts',(18.6098026989704,17.095124488636,-5.89512919840169));
#97758=CARTESIAN_POINT('Ctrl Pts',(18.8727052488065,17.0925251235231,-5.88065401520009));
#97759=CARTESIAN_POINT('Ctrl Pts',(19.0319913542557,17.1090085141082,-5.87222578061524));
#97760=CARTESIAN_POINT('Ctrl Pts',(19.2353088264538,17.1536389295898,-5.86047071503921));
#97761=CARTESIAN_POINT('Ctrl Pts',(19.2823439802619,17.165672836828,-5.8576758031864));
#97762=CARTESIAN_POINT('Ctrl Pts',(19.3363658020341,17.1814915286654,-5.8543339314129));
#97763=CARTESIAN_POINT('Ctrl Pts',(19.3437994995484,17.1837127088499,-5.85387113669538));
#97764=CARTESIAN_POINT('Ctrl Pts',(19.3556664474398,17.187329713356,-5.85312739536322));
#97765=CARTESIAN_POINT('Ctrl Pts',(19.3601076814325,17.1886993865335,-5.85284793585835));
#97766=CARTESIAN_POINT('Ctrl Pts',(19.3679697945519,17.1911524374952,-5.85235118897157));
#97767=CARTESIAN_POINT('Ctrl Pts',(19.3713924719027,17.1922299009648,-5.85213425011283));
#97768=CARTESIAN_POINT('Ctrl Pts',(19.3786459951136,17.1945336056696,-5.85167302430903));
#97769=CARTESIAN_POINT('Ctrl Pts',(19.3824760305682,17.1957620449101,-5.85142861507782));
#97770=CARTESIAN_POINT('Ctrl Pts',(19.3928137013193,17.1991102540189,-5.85076661869547));
#97771=CARTESIAN_POINT('Ctrl Pts',(19.3993145303316,17.2012506584647,-5.85034784518591));
#97772=CARTESIAN_POINT('Ctrl Pts',(19.431653329498,17.2120723375531,-5.84825266677946));
#97773=CARTESIAN_POINT('Ctrl Pts',(19.457331041608,17.2212201104345,-5.84655092681761));
#97774=CARTESIAN_POINT('Ctrl Pts',(19.5312425868864,17.249171022534,-5.84155577196845));
#97775=CARTESIAN_POINT('Ctrl Pts',(19.5789706385791,17.2692501247554,-5.83820915534393));
#97776=CARTESIAN_POINT('Ctrl Pts',(19.7513078878802,17.3493095465325,-5.82578780410558));
#97777=CARTESIAN_POINT('Ctrl Pts',(19.870706575776,17.4197130606724,-5.81654184700792));
#97778=CARTESIAN_POINT('Ctrl Pts',(20.0148091271497,17.5249309954341,-5.80498856794566));
#97779=CARTESIAN_POINT('Ctrl Pts',(20.0465534845629,17.5495234445017,-5.80241358872893));
#97780=CARTESIAN_POINT('Ctrl Pts',(20.1232167681151,17.6124840916443,-5.79612663753694));
#97781=CARTESIAN_POINT('Ctrl Pts',(20.1672677610612,17.6518589082214,-5.79245355201825));
#97782=CARTESIAN_POINT('Ctrl Pts',(20.2183872880876,17.7015521064076,-5.78811254465629));
#97783=CARTESIAN_POINT('Ctrl Pts',(20.2270825420895,17.7101525404416,-5.78737120593893));
#97784=CARTESIAN_POINT('Ctrl Pts',(20.2412898268673,17.7244505710342,-5.7861548676292));
#97785=CARTESIAN_POINT('Ctrl Pts',(20.246845164355,17.7301045484943,-5.78567795439805));
#97786=CARTESIAN_POINT('Ctrl Pts',(20.2568089909155,17.7403598738999,-5.78482016717834));
#97787=CARTESIAN_POINT('Ctrl Pts',(20.2612286863542,17.7449501562836,-5.78443880469588));
#97788=CARTESIAN_POINT('Ctrl Pts',(20.2706328865916,17.7548060083681,-5.78362543565624));
#97789=CARTESIAN_POINT('Ctrl Pts',(20.275611211643,17.760077381952,-5.78319369936979));
#97790=CARTESIAN_POINT('Ctrl Pts',(20.2890312644421,17.7744344515728,-5.78202662437894));
#97791=CARTESIAN_POINT('Ctrl Pts',(20.2974204768281,17.7835690101393,-5.78129353597302));
#97792=CARTESIAN_POINT('Ctrl Pts',(20.340155954464,17.8309301009973,-5.7775399555737));
#97793=CARTESIAN_POINT('Ctrl Pts',(20.3731839859538,17.8703261531367,-5.77457504135118));
#97794=CARTESIAN_POINT('Ctrl Pts',(20.5101843382777,18.0463824950438,-5.76191407953999));
#97795=CARTESIAN_POINT('Ctrl Pts',(20.5987432446707,18.1941924898872,-5.75281366859313));
#97796=CARTESIAN_POINT('Ctrl Pts',(20.7054257676578,18.4341850744421,-5.7383892691483));
#97797=CARTESIAN_POINT('Ctrl Pts',(20.7369711235795,18.5195786335076,-5.73330266197395));
#97798=CARTESIAN_POINT('Ctrl Pts',(20.7656831956612,18.6159825792187,-5.7273429922418));
#97799=CARTESIAN_POINT('Ctrl Pts',(20.7683774113313,18.6252604001434,-5.72676724776813));
#97800=CARTESIAN_POINT('Ctrl Pts',(20.7722640454593,18.6389947899297,-5.72591127197865));
#97801=CARTESIAN_POINT('Ctrl Pts',(20.7735055953079,18.6434374878978,-5.72563382137693));
#97802=CARTESIAN_POINT('Ctrl Pts',(20.7756835520062,18.6513304060546,-5.72513983980062));
#97803=CARTESIAN_POINT('Ctrl Pts',(20.7766257500082,18.6547789772849,-5.72492364859528));
#97804=CARTESIAN_POINT('Ctrl Pts',(20.7786269781943,18.6621774035352,-5.72445905031546));
#97805=CARTESIAN_POINT('Ctrl Pts',(20.7796832846299,18.6661278859382,-5.72421049542671));
#97806=CARTESIAN_POINT('Ctrl Pts',(20.7825542626137,18.6769910934836,-5.72352574716372));
#97807=CARTESIAN_POINT('Ctrl Pts',(20.7843453647729,18.6839099119624,-5.7230882273483));
#97808=CARTESIAN_POINT('Ctrl Pts',(20.7937636187623,18.7210660196281,-5.72073160698858));
#97809=CARTESIAN_POINT('Ctrl Pts',(20.8007565531057,18.7514582917134,-5.71877916700626));
#97810=CARTESIAN_POINT('Ctrl Pts',(20.8402826141576,18.9424582106662,-5.70640108722148));
#97811=CARTESIAN_POINT('Ctrl Pts',(20.8547462483627,19.106232430254,-5.69536328678664));
#97812=CARTESIAN_POINT('Ctrl Pts',(20.8469094631331,19.3871548150377,-5.67700409845332));
#97813=CARTESIAN_POINT('Ctrl Pts',(20.8339245839354,19.5038165535752,-5.66953962372299));
#97814=CARTESIAN_POINT('Ctrl Pts',(20.8085934887767,19.6328473343383,-5.66151057450884));
#97815=CARTESIAN_POINT('Ctrl Pts',(20.8056978483035,19.6468455669499,-5.66064231466571));
#97816=CARTESIAN_POINT('Ctrl Pts',(20.8008639227089,19.6690764416345,-5.65926764311523));
#97817=CARTESIAN_POINT('Ctrl Pts',(20.7990177406086,19.6773284631985,-5.65875830093279));
#97818=CARTESIAN_POINT('Ctrl Pts',(20.7956746885879,19.6918619037429,-5.65786282793587));
#97819=CARTESIAN_POINT('Ctrl Pts',(20.7941984389958,19.6981479091894,-5.65747604055645));
#97820=CARTESIAN_POINT('Ctrl Pts',(20.7910857781054,19.7111346590859,-5.6566779899948));
#97821=CARTESIAN_POINT('Ctrl Pts',(20.7894453299547,19.7178343644634,-5.65626686196399));
#97822=CARTESIAN_POINT('Ctrl Pts',(20.7851508707941,19.735009426156,-5.65521432959913));
#97823=CARTESIAN_POINT('Ctrl Pts',(20.7824493233422,19.7454727773353,-5.65457446554711));
#97824=CARTESIAN_POINT('Ctrl Pts',(20.7708431511412,19.789043547507,-5.6519152064258));
#97825=CARTESIAN_POINT('Ctrl Pts',(20.7612147880594,19.8219539790205,-5.64991930836331));
#97826=CARTESIAN_POINT('Ctrl Pts',(20.7340521654916,19.9070687127684,-5.64477911447693));
#97827=CARTESIAN_POINT('Ctrl Pts',(20.7152728911656,19.958849378079,-5.64167412969972));
#97828=CARTESIAN_POINT('Ctrl Pts',(20.653248441427,20.1110680065081,-5.63253421050392));
#97829=CARTESIAN_POINT('Ctrl Pts',(20.6042227374268,20.2089502977855,-5.62664802033573));
#97830=CARTESIAN_POINT('Ctrl Pts',(20.5264181760491,20.3382332752665,-5.61843315478145));
#97831=CARTESIAN_POINT('Ctrl Pts',(20.5039342831632,20.3732178105307,-5.61616062172462));
#97832=CARTESIAN_POINT('Ctrl Pts',(20.4369304437737,20.4710166000365,-5.60960323066978));
#97833=CARTESIAN_POINT('Ctrl Pts',(20.3899992829037,20.5320895511261,-5.60525798762717));
#97834=CARTESIAN_POINT('Ctrl Pts',(20.3336585315451,20.5976765936093,-5.60013372390642));
#97835=CARTESIAN_POINT('Ctrl Pts',(20.3274149299025,20.6048465648511,-5.59956702044052));
#97836=CARTESIAN_POINT('Ctrl Pts',(20.3180905126134,20.6154099298794,-5.59872196749233));
#97837=CARTESIAN_POINT('Ctrl Pts',(20.3150465321186,20.6188358802308,-5.59844629724577));
#97838=CARTESIAN_POINT('Ctrl Pts',(20.3096102484778,20.6249144615225,-5.59795427094486));
#97839=CARTESIAN_POINT('Ctrl Pts',(20.3072223324559,20.6275709484679,-5.59773824457235));
#97840=CARTESIAN_POINT('Ctrl Pts',(20.3020731900988,20.6332701404373,-5.59727261555843));
#97841=CARTESIAN_POINT('Ctrl Pts',(20.2993098662797,20.6363108095255,-5.59702285782825));
#97842=CARTESIAN_POINT('Ctrl Pts',(20.2916560429199,20.6446837175715,-5.59633147546365));
#97843=CARTESIAN_POINT('Ctrl Pts',(20.2867470854828,20.6499989003185,-5.59588848227961));
#97844=CARTESIAN_POINT('Ctrl Pts',(20.2596754155538,20.679010987308,-5.59344841529768));
#97845=CARTESIAN_POINT('Ctrl Pts',(20.2369986983407,20.7022197618821,-5.59141520590624));
#97846=CARTESIAN_POINT('Ctrl Pts',(20.0973928107142,20.8386812953483,-5.5790111528113));
#97847=CARTESIAN_POINT('Ctrl Pts',(19.968255172241,20.9386575017609,-5.56804893308317));
#97848=CARTESIAN_POINT('Ctrl Pts',(19.728948641116,21.0832755103828,-5.54978480276311));
#97849=CARTESIAN_POINT('Ctrl Pts',(19.6241156750034,21.1353285270644,-5.54234267676032));
#97850=CARTESIAN_POINT('Ctrl Pts',(19.5022235686276,21.1837457544456,-5.53433426640732));
#97851=CARTESIAN_POINT('Ctrl Pts',(19.4888876628176,21.1888872301853,-5.53346612303993));
#97852=CARTESIAN_POINT('Ctrl Pts',(19.4675807721743,21.1968549148413,-5.53209160046514));
#97853=CARTESIAN_POINT('Ctrl Pts',(19.459643334353,21.19976902798,-5.53158229177042));
#97854=CARTESIAN_POINT('Ctrl Pts',(19.4456140739619,21.2048244909252,-5.53068685772781));
#97855=CARTESIAN_POINT('Ctrl Pts',(19.4395295542947,21.206985656342,-5.53030007599484));
#97856=CARTESIAN_POINT('Ctrl Pts',(19.4269247980111,21.2113979111854,-5.52950201801098));
#97857=CARTESIAN_POINT('Ctrl Pts',(19.4204032490313,21.2136450409956,-5.52909087700565));
#97858=CARTESIAN_POINT('Ctrl Pts',(19.4036360509998,21.2193309873075,-5.52803827195416));
#97859=CARTESIAN_POINT('Ctrl Pts',(19.393374761598,21.2227233223537,-5.52739834860778));
#97860=CARTESIAN_POINT('Ctrl Pts',(19.3504470337057,21.2365512891226,-5.52473851341847));
#97861=CARTESIAN_POINT('Ctrl Pts',(19.3175543633144,21.2462713508712,-5.52274211157902));
#97862=CARTESIAN_POINT('Ctrl Pts',(19.2312560196539,21.2695089060162,-5.51760032715994));
#97863=CARTESIAN_POINT('Ctrl Pts',(19.1775324155649,21.2817491654307,-5.51449428753932));
#97864=CARTESIAN_POINT('Ctrl Pts',(19.0159315959175,21.3119890790746,-5.50535252786758));
#97865=CARTESIAN_POINT('Ctrl Pts',(18.9070745915923,21.3237438574571,-5.49946554599749));
#97866=CARTESIAN_POINT('Ctrl Pts',(18.7544583728296,21.3283451322055,-5.4911528179407));
#97867=CARTESIAN_POINT('Ctrl Pts',(18.7110908096744,21.3283199868743,-5.48878260171933));
#97868=CARTESIAN_POINT('Ctrl Pts',(18.6387100488214,21.3260539736983,-5.48477284606716));
#97869=CARTESIAN_POINT('Ctrl Pts',(18.6096869456578,21.3245466974369,-5.48315047434824));
#97870=CARTESIAN_POINT('Ctrl Pts',(18.5332573432183,21.3189977555048,-5.47881926008128));
#97871=CARTESIAN_POINT('Ctrl Pts',(18.4859430695756,21.3139548650726,-5.47607812533323));
#97872=CARTESIAN_POINT('Ctrl Pts',(18.4312003475133,21.3062472256842,-5.4727957736598));
#97873=CARTESIAN_POINT('Ctrl Pts',(18.4235638822542,21.3051294083639,-5.47233536967439));
#97874=CARTESIAN_POINT('Ctrl Pts',(18.4113506801935,21.3032733824279,-5.47159474472915));
#97875=CARTESIAN_POINT('Ctrl Pts',(18.4067698783917,21.3025618415347,-5.47131599126218));
#97876=CARTESIAN_POINT('Ctrl Pts',(18.3986490664127,21.3012730960857,-5.47082004350714));
#97877=CARTESIAN_POINT('Ctrl Pts',(18.3951081433952,21.3007019343047,-5.4706031938287));
#97878=CARTESIAN_POINT('Ctrl Pts',(18.3875926898239,21.2994700640224,-5.47014164207863));
#97879=CARTESIAN_POINT('Ctrl Pts',(18.3836186510041,21.2988070175452,-5.46989681511304));
#97880=CARTESIAN_POINT('Ctrl Pts',(18.3728689604189,21.2969819348036,-5.46923253297554));
#97881=CARTESIAN_POINT('Ctrl Pts',(18.3660971053576,21.295798243762,-5.46881187767169));
#97882=CARTESIAN_POINT('Ctrl Pts',(18.3321408619236,21.2896922465556,-5.46669201364089));
#97883=CARTESIAN_POINT('Ctrl Pts',(18.3050502688105,21.2842713718476,-5.46496676294433));
#97884=CARTESIAN_POINT('Ctrl Pts',(18.2265010432086,21.2669482138806,-5.45988011483574));
#97885=CARTESIAN_POINT('Ctrl Pts',(18.1753740442127,21.2536489017205,-5.45646335510192));
#97886=CARTESIAN_POINT('Ctrl Pts',(17.9780722831651,21.1943647012517,-5.44298866395169));
#97887=CARTESIAN_POINT('Ctrl Pts',(17.8365445792823,21.134471771628,-5.4327334595869));
#97888=CARTESIAN_POINT('Ctrl Pts',(17.6322552498939,21.0205186968665,-5.41770817525264));
#97889=CARTESIAN_POINT('Ctrl Pts',(17.5640878427914,20.9772127971188,-5.41264265204407));
#97890=CARTESIAN_POINT('Ctrl Pts',(17.4877036590849,20.9223190532456,-5.40690620733465));
#97891=CARTESIAN_POINT('Ctrl Pts',(17.4769290416364,20.9144201154912,-5.4060954528015));
#97892=CARTESIAN_POINT('Ctrl Pts',(17.4596772741709,20.9015198998366,-5.40479455543923));
#97893=CARTESIAN_POINT('Ctrl Pts',(17.4531532173695,20.8965822328406,-5.40430195153289));
#97894=CARTESIAN_POINT('Ctrl Pts',(17.441718210477,20.8878230359064,-5.40343733933386));
#97895=CARTESIAN_POINT('Ctrl Pts',(17.4367952091402,20.8840174682685,-5.40306470919026));
#97896=CARTESIAN_POINT('Ctrl Pts',(17.4265682941923,20.8760396008408,-5.40228975137037));
#97897=CARTESIAN_POINT('Ctrl Pts',(17.4212674012888,20.8718635294994,-5.40188757923018));
#97898=CARTESIAN_POINT('Ctrl Pts',(17.4076769412024,20.8610511803134,-5.40085516116281));
#97899=CARTESIAN_POINT('Ctrl Pts',(17.3994171083664,20.8543777002046,-5.40022641091924));
#97900=CARTESIAN_POINT('Ctrl Pts',(17.3815475914323,20.8397165552935,-5.3988631276667));
#97901=CARTESIAN_POINT('Ctrl Pts',(17.3719576744701,20.8317053551647,-5.39812956455156));
#97902=CARTESIAN_POINT('Ctrl Pts',(17.3443504457775,20.8082247831513,-5.39601157332466));
#97903=CARTESIAN_POINT('Ctrl Pts',(17.3265214507323,20.7925363064579,-5.39463596498888));
#97904=CARTESIAN_POINT('Ctrl Pts',(17.2657170197186,20.7371891588786,-5.38991166384915));
#97905=CARTESIAN_POINT('Ctrl Pts',(17.2241217530004,20.6960510723948,-5.38662221562829));
#97906=CARTESIAN_POINT('Ctrl Pts',(17.0705752943577,20.5310620699904,-5.37412313596597));
#97907=CARTESIAN_POINT('Ctrl Pts',(16.9717272268921,20.3958769292234,-5.36533455581101));
#97908=CARTESIAN_POINT('Ctrl Pts',(16.8619590343551,20.2011327200551,-5.35279638020422));
#97909=CARTESIAN_POINT('Ctrl Pts',(16.8361298907681,20.1506744272087,-5.3495523903727));
#97910=CARTESIAN_POINT('Ctrl Pts',(16.8086457512731,20.0912149151449,-5.34566616102009));
#97911=CARTESIAN_POINT('Ctrl Pts',(16.8049839540475,20.083160746777,-5.34513842711246));
#97912=CARTESIAN_POINT('Ctrl Pts',(16.7995317710099,20.0709662878449,-5.34433707457302));
#97913=CARTESIAN_POINT('Ctrl Pts',(16.7977039031392,20.0668427248148,-5.34406569607154));
#97914=CARTESIAN_POINT('Ctrl Pts',(16.7944546135634,20.0594488255301,-5.34357832025268));
#97915=CARTESIAN_POINT('Ctrl Pts',(16.7930282644025,20.0561807125852,-5.34336262825377));
#97916=CARTESIAN_POINT('Ctrl Pts',(16.7899560464386,20.0490927195048,-5.34289422821695));
#97917=CARTESIAN_POINT('Ctrl Pts',(16.7883131984231,20.0452716400236,-5.34264134642966));
#97918=CARTESIAN_POINT('Ctrl Pts',(16.7837528404042,20.0345780232952,-5.34193265037776));
#97919=CARTESIAN_POINT('Ctrl Pts',(16.7808604447694,20.0276949356661,-5.34147535494318));
#97920=CARTESIAN_POINT('Ctrl Pts',(16.764222646662,19.9875077471839,-5.3387994386588));
#97921=CARTESIAN_POINT('Ctrl Pts',(16.7512937136483,19.9538745029651,-5.33653614540452));
#97922=CARTESIAN_POINT('Ctrl Pts',(16.7123940719146,19.8444196762135,-5.32913131005087));
#97923=CARTESIAN_POINT('Ctrl Pts',(16.6898690219549,19.7674511146764,-5.32386679432088));
#97924=CARTESIAN_POINT('Ctrl Pts',(16.6354601235266,19.5329093389116,-5.30797072274112));
#97925=CARTESIAN_POINT('Ctrl Pts',(16.6170836488932,19.3727774115619,-5.2973580198773));
#97926=CARTESIAN_POINT('Ctrl Pts',(16.617000284924,19.2120983478179,-5.28730622481232));
#97927=CARTESIAN_POINT('Ctrl Pts',(16.6170002837517,19.2120960860112,-5.28730608331776));
#97928=CARTESIAN_POINT('Ctrl Pts',(16.6169868618999,19.1861728863881,-5.28568437508849));
#97929=CARTESIAN_POINT('Ctrl Pts',(16.6174495936717,19.160250559852,-5.28407668349347));
#97930=CARTESIAN_POINT('Ctrl Pts',(16.619026332341,19.1167355687962,-5.28140090887606));
#97931=CARTESIAN_POINT('Ctrl Pts',(16.6198840725551,19.0991372597741,-5.28032509221211));
#97932=CARTESIAN_POINT('Ctrl Pts',(16.6214584305574,19.0734384407885,-5.27876299621345));
#97933=CARTESIAN_POINT('Ctrl Pts',(16.6220021625087,19.0653284430094,-5.27827133051497));
#97934=CARTESIAN_POINT('Ctrl Pts',(16.62304733721,19.050977982414,-5.27740358656125));
#97935=CARTESIAN_POINT('Ctrl Pts',(16.6235297763263,19.0447362728896,-5.27702691609314));
#97936=CARTESIAN_POINT('Ctrl Pts',(16.6245388687024,19.0323936384307,-5.27628353155207));
#97937=CARTESIAN_POINT('Ctrl Pts',(16.6250643196937,19.0262926790796,-5.27591678345692));
#97938=CARTESIAN_POINT('Ctrl Pts',(16.6261638693465,19.0141427830512,-5.27518779097605));
#97939=CARTESIAN_POINT('Ctrl Pts',(16.6267375529903,19.0080938685996,-5.27482553722127));
#97940=CARTESIAN_POINT('Ctrl Pts',(16.6281714449769,18.9936373475952,-5.2739613605212));
#97941=CARTESIAN_POINT('Ctrl Pts',(16.6290559777756,18.9852322160711,-5.27346020631224));
#97942=CARTESIAN_POINT('Ctrl Pts',(16.6319011555824,18.9596681197253,-5.27193970990869));
#97943=CARTESIAN_POINT('Ctrl Pts',(16.634021488887,18.9425273855968,-5.27092538153886));
#97944=CARTESIAN_POINT('Ctrl Pts',(16.6419662052317,18.8841728758714,-5.26748807325364));
#97945=CARTESIAN_POINT('Ctrl Pts',(16.6487962821945,18.8431044315344,-5.26509633856523));
#97946=CARTESIAN_POINT('Ctrl Pts',(16.6780901108046,18.6942360310667,-5.25649241599256));
#97947=CARTESIAN_POINT('Ctrl Pts',(16.7077221576858,18.5881302047764,-5.25049678412355));
#97948=CARTESIAN_POINT('Ctrl Pts',(16.745419381199,18.4848897311503,-5.24452701096005));
#97949=CARTESIAN_POINT('Origin',(18.734,19.211,0.));
#97950=CARTESIAN_POINT('',(16.7454194484637,18.4848895469342,-4.44630497835508));
#97951=CARTESIAN_POINT('',(16.7454194645813,18.4848895027932,-4.66702131702538));
#97952=CARTESIAN_POINT('',(16.7454194503191,18.4848895418526,0.));
#97953=CARTESIAN_POINT('Ctrl Pts',(16.7454194645813,18.4848895027932,-4.66702131702538));
#97954=CARTESIAN_POINT('Ctrl Pts',(16.6988234574177,18.6125008143362,-4.67446195852453));
#97955=CARTESIAN_POINT('Ctrl Pts',(16.66461025224,18.744325088795,-4.68169548026336));
#97956=CARTESIAN_POINT('Ctrl Pts',(16.6370543938698,18.9176173124031,-4.69152882229505));
#97957=CARTESIAN_POINT('Ctrl Pts',(16.6319381925939,18.9568542403389,-4.69377779250457));
#97958=CARTESIAN_POINT('Ctrl Pts',(16.6263939805864,19.0112165310485,-4.69695244130703));
#97959=CARTESIAN_POINT('Ctrl Pts',(16.6250239202028,19.0262395182405,-4.69783592543835));
#97960=CARTESIAN_POINT('Ctrl Pts',(16.6229323256568,19.0522443093919,-4.69937786513208));
#97961=CARTESIAN_POINT('Ctrl Pts',(16.6221356455648,19.0632196503181,-4.70003252474882));
#97962=CARTESIAN_POINT('Ctrl Pts',(16.6211102620339,19.0790544965181,-4.70098327938888));
#97963=CARTESIAN_POINT('Ctrl Pts',(16.6208126722696,19.0839095694667,-4.701275631674));
#97964=CARTESIAN_POINT('Ctrl Pts',(16.6203235174211,19.0923671963612,-4.70178645165111));
#97965=CARTESIAN_POINT('Ctrl Pts',(16.6201244222695,19.0959693221627,-4.70200449766765));
#97966=CARTESIAN_POINT('Ctrl Pts',(16.6197264096915,19.1035206041751,-4.70246264082655));
#97967=CARTESIAN_POINT('Ctrl Pts',(16.6195293494629,19.10746979848,-4.70270283607585));
#97968=CARTESIAN_POINT('Ctrl Pts',(16.6190357978279,19.1179506865753,-4.70334183187577));
#97969=CARTESIAN_POINT('Ctrl Pts',(16.6187585034882,19.1244831805591,-4.70374168383773));
#97970=CARTESIAN_POINT('Ctrl Pts',(16.6177066684856,19.1523033179473,-4.70545097380983));
#97971=CARTESIAN_POINT('Ctrl Pts',(16.6172232245839,19.1735998901574,-4.70677546541417));
#97972=CARTESIAN_POINT('Ctrl Pts',(16.6170218767773,19.200073104592,-4.70843882601727));
#97973=CARTESIAN_POINT('Ctrl Pts',(16.6170014935553,19.2052471239773,-4.70876472284575));
#97974=CARTESIAN_POINT('Ctrl Pts',(16.6169868171449,19.2589278692597,-4.71215391036776));
#97975=CARTESIAN_POINT('Ctrl Pts',(16.6186407108918,19.3074176155505,-4.71528275379712));
#97976=CARTESIAN_POINT('Ctrl Pts',(16.6353861331744,19.5516577913175,-4.73125346316285));
#97977=CARTESIAN_POINT('Ctrl Pts',(16.6759975066366,19.7447399354121,-4.74444610218463));
#97978=CARTESIAN_POINT('Ctrl Pts',(16.7587957145083,19.9742314962044,-4.75978159654064));
#97979=CARTESIAN_POINT('Ctrl Pts',(16.7764544915404,20.0184468654001,-4.76272638402557));
#97980=CARTESIAN_POINT('Ctrl Pts',(16.8006203653444,20.0734898657946,-4.7663823368788));
#97981=CARTESIAN_POINT('Ctrl Pts',(16.8057522324957,20.0849028195151,-4.76713986251815));
#97982=CARTESIAN_POINT('Ctrl Pts',(16.8140577645003,20.1029443951343,-4.76833669134979));
#97983=CARTESIAN_POINT('Ctrl Pts',(16.8171652094914,20.1096030156214,-4.76877826123794));
#97984=CARTESIAN_POINT('Ctrl Pts',(16.823028055914,20.1219970985968,-4.76959995815116));
#97985=CARTESIAN_POINT('Ctrl Pts',(16.8257747608685,20.1277365613108,-4.76998038042889));
#97986=CARTESIAN_POINT('Ctrl Pts',(16.8319433128508,20.1404784015904,-4.77082477432642));
#97987=CARTESIAN_POINT('Ctrl Pts',(16.8353780471961,20.1474744646648,-4.77128829154419));
#97988=CARTESIAN_POINT('Ctrl Pts',(16.8455036889344,20.1678142453384,-4.77263567946622));
#97989=CARTESIAN_POINT('Ctrl Pts',(16.8522972737284,20.1811065322949,-4.77351595259198));
#97990=CARTESIAN_POINT('Ctrl Pts',(16.9092402101685,20.289671584962,-4.78070597854901));
#97991=CARTESIAN_POINT('Ctrl Pts',(16.9664529731369,20.3810694934547,-4.78674993048902));
#97992=CARTESIAN_POINT('Ctrl Pts',(17.1097563341115,20.5753316980448,-4.80001601635743));
#97993=CARTESIAN_POINT('Ctrl Pts',(17.1991453836981,20.6751676246587,-4.80713510492787));
#97994=CARTESIAN_POINT('Ctrl Pts',(17.3094007822207,20.7770381047402,-4.81548127362692));
#97995=CARTESIAN_POINT('Ctrl Pts',(17.3215822631169,20.7880334155392,-4.81639837091414));
#97996=CARTESIAN_POINT('Ctrl Pts',(17.373692197529,20.8339810742921,-4.8203064141723));
#97997=CARTESIAN_POINT('Ctrl Pts',(17.4147963007586,20.8675643603935,-4.82335196781879));
#97998=CARTESIAN_POINT('Ctrl Pts',(17.4640569638761,20.904815056129,-4.82701707430932));
#97999=CARTESIAN_POINT('Ctrl Pts',(17.4710316282704,20.910021967337,-4.82753635032579));
#98000=CARTESIAN_POINT('Ctrl Pts',(17.481644252569,20.9178433290356,-4.8283273311095));
#98001=CARTESIAN_POINT('Ctrl Pts',(17.4852588266247,20.9204895580453,-4.82859688115313));
#98002=CARTESIAN_POINT('Ctrl Pts',(17.4917639171662,20.9252202935484,-4.82908230549878));
#98003=CARTESIAN_POINT('Ctrl Pts',(17.4946513198195,20.9273089899384,-4.82929788489472));
#98004=CARTESIAN_POINT('Ctrl Pts',(17.5009390504933,20.9318332832327,-4.82976760082909));
#98005=CARTESIAN_POINT('Ctrl Pts',(17.5043412822405,20.9342660650693,-4.83002191959921));
#98006=CARTESIAN_POINT('Ctrl Pts',(17.5139239269522,20.9410753531651,-4.83073862393211));
#98007=CARTESIAN_POINT('Ctrl Pts',(17.5201205743176,20.9454287496401,-4.8312025441027));
#98008=CARTESIAN_POINT('Ctrl Pts',(17.5574253897987,20.9713390609635,-4.83399751539601));
#98009=CARTESIAN_POINT('Ctrl Pts',(17.5890816778356,20.9920904097943,-4.83637790462689));
#98010=CARTESIAN_POINT('Ctrl Pts',(17.6953709858567,21.0577606335277,-4.84435490029763));
#98011=CARTESIAN_POINT('Ctrl Pts',(17.7722173269281,21.0989214065626,-4.85009463079852));
#98012=CARTESIAN_POINT('Ctrl Pts',(18.0107243942808,21.2083222871105,-4.86743182627381));
#98013=CARTESIAN_POINT('Ctrl Pts',(18.1785701436342,21.2613524066277,-4.87894125133019));
#98014=CARTESIAN_POINT('Ctrl Pts',(18.3736794421063,21.2972375609875,-4.89115214668771));
#98015=CARTESIAN_POINT('Ctrl Pts',(18.3963683895905,21.3010294319637,-4.89255631343321));
#98016=CARTESIAN_POINT('Ctrl Pts',(18.4285569776615,21.3058710512096,-4.89452676420059));
#98017=CARTESIAN_POINT('Ctrl Pts',(18.4380082189428,21.3072273329269,-4.89510270707347));
#98018=CARTESIAN_POINT('Ctrl Pts',(18.4533806355021,21.3093272811114,-4.89603530195001));
#98019=CARTESIAN_POINT('Ctrl Pts',(18.4592962704175,21.3101099229136,-4.89639318218107));
#98020=CARTESIAN_POINT('Ctrl Pts',(18.4716866219836,21.3116958983636,-4.89714069867419));
#98021=CARTESIAN_POINT('Ctrl Pts',(18.4781619108412,21.312494334823,-4.89753017659066));
#98022=CARTESIAN_POINT('Ctrl Pts',(18.4935764075615,21.3143227198565,-4.89845457704296));
#98023=CARTESIAN_POINT('Ctrl Pts',(18.5025187409409,21.3153256397661,-4.89898864230417));
#98024=CARTESIAN_POINT('Ctrl Pts',(18.5326722001821,21.318512939129,-4.9007822924993));
#98025=CARTESIAN_POINT('Ctrl Pts',(18.5539102921976,21.3204339092809,-4.90203359417181));
#98026=CARTESIAN_POINT('Ctrl Pts',(18.6697208013014,21.3291470229912,-4.90879675696166));
#98027=CARTESIAN_POINT('Ctrl Pts',(18.7646440373952,21.3299012721082,-4.91411544545084));
#98028=CARTESIAN_POINT('Ctrl Pts',(19.0284622397008,21.3142581753223,-4.92865689622046));
#98029=CARTESIAN_POINT('Ctrl Pts',(19.1957807525193,21.2839568251217,-4.9375737220549));
#98030=CARTESIAN_POINT('Ctrl Pts',(19.3942231775491,21.2227794841407,-4.94941672400651));
#98031=CARTESIAN_POINT('Ctrl Pts',(19.4304520589743,21.2105263083619,-4.95163553070747));
#98032=CARTESIAN_POINT('Ctrl Pts',(19.4731095581262,21.1947989623043,-4.9543379330653));
#98033=CARTESIAN_POINT('Ctrl Pts',(19.4798795018202,21.1922634926047,-4.95476954671575));
#98034=CARTESIAN_POINT('Ctrl Pts',(19.4908786137344,21.188079757111,-4.95547544488958));
#98035=CARTESIAN_POINT('Ctrl Pts',(19.4951157652467,21.1864524527102,-4.95574850559991));
#98036=CARTESIAN_POINT('Ctrl Pts',(19.502674395544,21.1835215854793,-4.95623769310054));
#98037=CARTESIAN_POINT('Ctrl Pts',(19.5059978417334,21.1822232404395,-4.9564535050126));
#98038=CARTESIAN_POINT('Ctrl Pts',(19.5131693283762,21.1794006928996,-4.95692076825145));
#98039=CARTESIAN_POINT('Ctrl Pts',(19.5170161318849,21.1778736275167,-4.95717238581413));
#98040=CARTESIAN_POINT('Ctrl Pts',(19.5277027373964,21.1735950470494,-4.95787406001067));
#98041=CARTESIAN_POINT('Ctrl Pts',(19.5345326039404,21.1708190988973,-4.95832555166087));
#98042=CARTESIAN_POINT('Ctrl Pts',(19.5732605924124,21.1548421791802,-4.9609024645476));
#98043=CARTESIAN_POINT('Ctrl Pts',(19.6048445963251,21.1408989949771,-4.96306886047731));
#98044=CARTESIAN_POINT('Ctrl Pts',(19.7036377744781,21.0943665572877,-4.97002075292179));
#98045=CARTESIAN_POINT('Ctrl Pts',(19.7694682536341,21.0589910621757,-4.97491417818913));
#98046=CARTESIAN_POINT('Ctrl Pts',(19.9991769554074,20.9194189890758,-4.99264212121274));
#98047=CARTESIAN_POINT('Ctrl Pts',(20.1504570886518,20.7962599464977,-5.00546980764393));
#98048=CARTESIAN_POINT('Ctrl Pts',(20.2972438308747,20.6387269067766,-5.01869840151999));
#98049=CARTESIAN_POINT('Ctrl Pts',(20.31141526599,20.6230540090637,-5.01998660102361));
#98050=CARTESIAN_POINT('Ctrl Pts',(20.3308238122341,20.6009322278203,-5.02176706530472));
#98051=CARTESIAN_POINT('Ctrl Pts',(20.3362608343112,20.5946611243915,-5.02226766467881));
#98052=CARTESIAN_POINT('Ctrl Pts',(20.3455882459795,20.5837741120739,-5.02312969880941));
#98053=CARTESIAN_POINT('Ctrl Pts',(20.3494960018881,20.5791732735355,-5.02349184969312));
#98054=CARTESIAN_POINT('Ctrl Pts',(20.3575532343649,20.569604355026,-5.02424066262373));
#98055=CARTESIAN_POINT('Ctrl Pts',(20.3616997154676,20.564633826415,-5.02462719957479));
#98056=CARTESIAN_POINT('Ctrl Pts',(20.3713673559584,20.5529362412866,-5.02553124212869));
#98057=CARTESIAN_POINT('Ctrl Pts',(20.3768699878682,20.5461939710943,-5.02604799180047));
#98058=CARTESIAN_POINT('Ctrl Pts',(20.3946453041218,20.5241379567078,-5.02772461082035));
#98059=CARTESIAN_POINT('Ctrl Pts',(20.4067468875821,20.5086871764136,-5.02887762130791));
#98060=CARTESIAN_POINT('Ctrl Pts',(20.4678027198295,20.4284601815563,-5.03475909175496));
#98061=CARTESIAN_POINT('Ctrl Pts',(20.5132187216919,20.3610712973861,-5.03934822491166));
#98062=CARTESIAN_POINT('Ctrl Pts',(20.6406813700746,20.1462423227603,-5.05319189609479));
#98063=CARTESIAN_POINT('Ctrl Pts',(20.7090724430763,19.9915082600914,-5.0620626918143));
#98064=CARTESIAN_POINT('Ctrl Pts',(20.7741263764752,19.7788629866068,-5.07456389136168));
#98065=CARTESIAN_POINT('Ctrl Pts',(20.7878981153823,19.7268347526823,-5.07765029257518));
#98066=CARTESIAN_POINT('Ctrl Pts',(20.8015844539561,19.6658184894189,-5.08136102593395));
#98067=CARTESIAN_POINT('Ctrl Pts',(20.8034438411121,19.6572818785142,-5.08188223772846));
#98068=CARTESIAN_POINT('Ctrl Pts',(20.8061780396652,19.6443443242729,-5.0826755933476));
#98069=CARTESIAN_POINT('Ctrl Pts',(20.8070918134197,19.6399515866976,-5.08294556303785));
#98070=CARTESIAN_POINT('Ctrl Pts',(20.8087063952332,19.6320642198032,-5.08343143358339));
#98071=CARTESIAN_POINT('Ctrl Pts',(20.8094123481887,19.6285706985794,-5.08364703714067));
#98072=CARTESIAN_POINT('Ctrl Pts',(20.8109265117657,19.6209789179596,-5.08411644344029));
#98073=CARTESIAN_POINT('Ctrl Pts',(20.8117314055249,19.6168800983621,-5.08437042643753));
#98074=CARTESIAN_POINT('Ctrl Pts',(20.8139566794485,19.6053680830238,-5.08508525680834));
#98075=CARTESIAN_POINT('Ctrl Pts',(20.8153495340956,19.5979497205955,-5.08554762620798));
#98076=CARTESIAN_POINT('Ctrl Pts',(20.8234096700197,19.5537183734045,-5.08831411978127));
#98077=CARTESIAN_POINT('Ctrl Pts',(20.8291393770273,19.5167437584401,-5.09066644425214));
#98078=CARTESIAN_POINT('Ctrl Pts',(20.8447218636128,19.3949394702345,-5.0985036897849));
#98079=CARTESIAN_POINT('Ctrl Pts',(20.8504223412073,19.3096666831819,-5.10412669952517));
#98080=CARTESIAN_POINT('Ctrl Pts',(20.852074192631,19.0465236464045,-5.1215109985812));
#98081=CARTESIAN_POINT('Ctrl Pts',(20.8307946317997,18.8692875652443,-5.13319192669085));
#98082=CARTESIAN_POINT('Ctrl Pts',(20.7820564236979,18.6746472374158,-5.14554011528105));
#98083=CARTESIAN_POINT('Ctrl Pts',(20.776157785983,18.652608522954,-5.14693256727195));
#98084=CARTESIAN_POINT('Ctrl Pts',(20.7672950736057,18.6215165718268,-5.1488895816805));
#98085=CARTESIAN_POINT('Ctrl Pts',(20.7646245401782,18.6123819666164,-5.14946362526579));
#98086=CARTESIAN_POINT('Ctrl Pts',(20.7601810820551,18.5975550048967,-5.15039398496426));
#98087=CARTESIAN_POINT('Ctrl Pts',(20.7584455711271,18.5918516575419,-5.15075151766503));
#98088=CARTESIAN_POINT('Ctrl Pts',(20.7547588473058,18.5799173496861,-5.1514989748786));
#98089=CARTESIAN_POINT('Ctrl Pts',(20.7528028505029,18.5736879235679,-5.15188873811846));
#98090=CARTESIAN_POINT('Ctrl Pts',(20.7480744607896,18.5588692421862,-5.15281502934689));
#98091=CARTESIAN_POINT('Ctrl Pts',(20.7452758833745,18.5502884262482,-5.15335069059783));
#98092=CARTESIAN_POINT('Ctrl Pts',(20.7356303210785,18.5213430995984,-5.1551554123184));
#98093=CARTESIAN_POINT('Ctrl Pts',(20.7285280991241,18.5010645843888,-5.15641604732768));
#98094=CARTESIAN_POINT('Ctrl Pts',(20.6593418037715,18.3127605060513,-5.16809653375303));
#98095=CARTESIAN_POINT('Ctrl Pts',(20.5764785248977,18.1531459692136,-5.17772287233326));
#98096=CARTESIAN_POINT('Ctrl Pts',(20.40570003958,17.9065028038249,-5.19404858118146));
#98097=CARTESIAN_POINT('Ctrl Pts',(20.328531478131,17.8132322136214,-5.20067729948763));
#98098=CARTESIAN_POINT('Ctrl Pts',(20.2371952744552,17.720301187994,-5.2083999392276));
#98099=CARTESIAN_POINT('Ctrl Pts',(20.2305008150659,17.7135807920984,-5.2089653677263));
#98100=CARTESIAN_POINT('Ctrl Pts',(20.2205084800376,17.7036836751694,-5.20980887927629));
#98101=CARTESIAN_POINT('Ctrl Pts',(20.2172449913798,17.7004721919251,-5.21008429725847));
#98102=CARTESIAN_POINT('Ctrl Pts',(20.2114172864118,17.6947744499762,-5.21057604772473));
#98103=CARTESIAN_POINT('Ctrl Pts',(20.2088571714755,17.6922840686129,-5.21079205195714));
#98104=CARTESIAN_POINT('Ctrl Pts',(20.2033362946632,17.6869406972459,-5.21125783251008));
#98105=CARTESIAN_POINT('Ctrl Pts',(20.2003735633168,17.6840898922113,-5.21150776497149));
#98106=CARTESIAN_POINT('Ctrl Pts',(20.1921650037943,17.6762373610213,-5.21220011231284));
#98107=CARTESIAN_POINT('Ctrl Pts',(20.1869018216996,17.671253972469,-5.21264390191453));
#98108=CARTESIAN_POINT('Ctrl Pts',(20.1578012249538,17.6439824317191,-5.21509640628565));
#98109=CARTESIAN_POINT('Ctrl Pts',(20.1334778715711,17.6222220409873,-5.21714168342497));
#98110=CARTESIAN_POINT('Ctrl Pts',(19.9849903831066,17.4954366051412,-5.22954980491163));
#98111=CARTESIAN_POINT('Ctrl Pts',(19.8495662594593,17.4044434511716,-5.24050098099606));
#98112=CARTESIAN_POINT('Ctrl Pts',(19.6012509177667,17.2762614295174,-5.25875414881715));
#98113=CARTESIAN_POINT('Ctrl Pts',(19.493169104198,17.2313516544784,-5.26619577951411));
#98114=CARTESIAN_POINT('Ctrl Pts',(19.3683366318617,17.191220430012,-5.27420198193072));
#98115=CARTESIAN_POINT('Ctrl Pts',(19.3547126667837,17.1869920269941,-5.27506842393795));
#98116=CARTESIAN_POINT('Ctrl Pts',(19.3329541855649,17.1804793179396,-5.27644077026794));
#98117=CARTESIAN_POINT('Ctrl Pts',(19.3248471184224,17.1781055013691,-5.27694958966385));
#98118=CARTESIAN_POINT('Ctrl Pts',(19.3105198097889,17.1740032933581,-5.27784445474815));
#98119=CARTESIAN_POINT('Ctrl Pts',(19.3043055045365,17.1722547224147,-5.27823115419692));
#98120=CARTESIAN_POINT('Ctrl Pts',(19.2914317294757,17.1686957888675,-5.27902932161128));
#98121=CARTESIAN_POINT('Ctrl Pts',(19.2847712036161,17.1668895071848,-5.2794406529545));
#98122=CARTESIAN_POINT('Ctrl Pts',(19.2676433850478,17.1623343721844,-5.28049432387994));
#98123=CARTESIAN_POINT('Ctrl Pts',(19.2571635494368,17.1596331327328,-5.28113511663186));
#98124=CARTESIAN_POINT('Ctrl Pts',(19.2132658537066,17.1486765245523,-5.28380341199279));
#98125=CARTESIAN_POINT('Ctrl Pts',(19.1796687738439,17.1411561850023,-5.2858072132766));
#98126=CARTESIAN_POINT('Ctrl Pts',(19.0915961329795,17.1236861415526,-5.29097237850196));
#98127=CARTESIAN_POINT('Ctrl Pts',(19.036886377878,17.1150480365207,-5.29409392857891));
#98128=CARTESIAN_POINT('Ctrl Pts',(18.8730906016543,17.095734913275,-5.30326273946136));
#98129=CARTESIAN_POINT('Ctrl Pts',(18.7634487630281,17.0913712090237,-5.3091613544561));
#98130=CARTESIAN_POINT('Ctrl Pts',(18.5936323344809,17.0977960734939,-5.31841466959183));
#98131=CARTESIAN_POINT('Ctrl Pts',(18.5334302117375,17.1026582291857,-5.32172055381736));
#98132=CARTESIAN_POINT('Ctrl Pts',(18.4157446272804,17.1172493075713,-5.32836359578313));
#98133=CARTESIAN_POINT('Ctrl Pts',(18.3582935058201,17.1267922885538,-5.33169277155115));
#98134=CARTESIAN_POINT('Ctrl Pts',(18.2925983050441,17.1405090374674,-5.33567393163575));
#98135=CARTESIAN_POINT('Ctrl Pts',(18.2838939502995,17.1423838393813,-5.33620499030984));
#98136=CARTESIAN_POINT('Ctrl Pts',(18.2707867154551,17.1452936057689,-5.33701041681783));
#98137=CARTESIAN_POINT('Ctrl Pts',(18.2663747752304,17.1462878887279,-5.33728251052522));
#98138=CARTESIAN_POINT('Ctrl Pts',(18.2584890838033,17.148091594195,-5.33777065477873));
#98139=CARTESIAN_POINT('Ctrl Pts',(18.2550141624138,17.1488956647912,-5.33798639594007));
#98140=CARTESIAN_POINT('Ctrl Pts',(18.2474999580234,17.1506544134868,-5.33845430438067));
#98141=CARTESIAN_POINT('Ctrl Pts',(18.2434615014439,17.1516121765294,-5.33870664218224));
#98142=CARTESIAN_POINT('Ctrl Pts',(18.2322055765157,17.1543166262999,-5.33941231404738));
#98143=CARTESIAN_POINT('Ctrl Pts',(18.2249945255667,17.1560894018634,-5.33986710932274));
#98144=CARTESIAN_POINT('Ctrl Pts',(18.1834902308312,17.1665247459197,-5.34249979479707));
#98145=CARTESIAN_POINT('Ctrl Pts',(18.1494111881358,17.1760072109599,-5.3447207224182));
#98146=CARTESIAN_POINT('Ctrl Pts',(18.0412567969326,17.2090418452874,-5.35192534350078));
#98147=CARTESIAN_POINT('Ctrl Pts',(17.9682370295545,17.2358202525296,-5.35702525829945));
#98148=CARTESIAN_POINT('Ctrl Pts',(17.7268424049412,17.3397473451085,-5.37436991876636));
#98149=CARTESIAN_POINT('Ctrl Pts',(17.5671202279576,17.4349449970406,-5.38658847261831));
#98150=CARTESIAN_POINT('Ctrl Pts',(17.4024246351647,17.5650334089522,-5.39952828948029));
#98151=CARTESIAN_POINT('Ctrl Pts',(17.3833124394935,17.580680348512,-5.40103764730808));
#98152=CARTESIAN_POINT('Ctrl Pts',(17.3569790414246,17.603020217905,-5.40312909352447));
#98153=CARTESIAN_POINT('Ctrl Pts',(17.3495246306124,17.6094339986604,-5.40372249904741));
#98154=CARTESIAN_POINT('Ctrl Pts',(17.337579317074,17.6198574814043,-5.40467570042938));
#98155=CARTESIAN_POINT('Ctrl Pts',(17.3330604201126,17.6238347493549,-5.40503683318622));
#98156=CARTESIAN_POINT('Ctrl Pts',(17.3240070515465,17.6318717826441,-5.40576145854981));
#98157=CARTESIAN_POINT('Ctrl Pts',(17.3194729994174,17.6359319356438,-5.40612492990108));
#98158=CARTESIAN_POINT('Ctrl Pts',(17.3087575434609,17.6456110004192,-5.40698532677446));
#98159=CARTESIAN_POINT('Ctrl Pts',(17.3025917338053,17.6512470841663,-5.40748152144987));
#98160=CARTESIAN_POINT('Ctrl Pts',(17.2833844706732,17.6690140031828,-5.4090308788075));
#98161=CARTESIAN_POINT('Ctrl Pts',(17.2704624312886,17.6812732132746,-5.41007855568076));
#98162=CARTESIAN_POINT('Ctrl Pts',(17.2407218398731,17.7102101273218,-5.41250363177934));
#98163=CARTESIAN_POINT('Ctrl Pts',(17.2240252300558,17.7270100529576,-5.4138756822937));
#98164=CARTESIAN_POINT('Ctrl Pts',(17.1672501941593,17.786086938513,-5.4185839250987));
#98165=CARTESIAN_POINT('Ctrl Pts',(17.1286356377501,17.8297367398963,-5.42186133841043));
#98166=CARTESIAN_POINT('Ctrl Pts',(16.9872885638627,18.0034625625894,-5.43428376472812));
#98167=CARTESIAN_POINT('Ctrl Pts',(16.8981704334622,18.1438211181074,-5.4430137233738));
#98168=CARTESIAN_POINT('Ctrl Pts',(16.8011345781242,18.3454955232621,-5.45555189605258));
#98169=CARTESIAN_POINT('Ctrl Pts',(16.7781056627413,18.3988775980773,-5.45887555300619));
#98170=CARTESIAN_POINT('Ctrl Pts',(16.7541175175169,18.4614444156118,-5.46285056196539));
#98171=CARTESIAN_POINT('Ctrl Pts',(16.7509837343203,18.4697748639589,-5.46338140995003));
#98172=CARTESIAN_POINT('Ctrl Pts',(16.7470710655027,18.4803782241668,-5.46405941616438));
#98173=CARTESIAN_POINT('Ctrl Pts',(16.7462433354765,18.4826331881799,-5.46420373713071));
#98174=CARTESIAN_POINT('Ctrl Pts',(16.7454194503191,18.4848895418527,-5.46434828430915));
#98175=CARTESIAN_POINT('Ctrl Pts',(16.745419381199,18.4848897311503,-5.24452701096005));
#98176=CARTESIAN_POINT('Ctrl Pts',(16.7665875207388,18.4269170597383,-5.24117480144515));
#98177=CARTESIAN_POINT('Ctrl Pts',(16.79029877288,18.369848040943,-5.23782816810057));
#98178=CARTESIAN_POINT('Ctrl Pts',(16.8430672123269,18.2570645705659,-5.23098482960947));
#98179=CARTESIAN_POINT('Ctrl Pts',(16.8721437363652,18.2014903584518,-5.2274929886192));
#98180=CARTESIAN_POINT('Ctrl Pts',(16.9191780061591,18.1205568161515,-5.22210863810526));
#98181=CARTESIAN_POINT('Ctrl Pts',(16.9352983715831,18.0941663366885,-5.22030283547618));
#98182=CARTESIAN_POINT('Ctrl Pts',(16.9558380197945,18.062139789975,-5.21803691042424));
#98183=CARTESIAN_POINT('Ctrl Pts',(16.9597163424726,18.0561591844035,-5.21761051195919));
#98184=CARTESIAN_POINT('Ctrl Pts',(16.9658647108679,18.0467821133109,-5.21693661899035));
#98185=CARTESIAN_POINT('Ctrl Pts',(16.9681145521063,18.043372374158,-5.21669045644307));
#98186=CARTESIAN_POINT('Ctrl Pts',(16.9723521719804,18.0369903254211,-5.21622756791302));
#98187=CARTESIAN_POINT('Ctrl Pts',(16.9743376167164,18.0340165327635,-5.21601099811852));
#98188=CARTESIAN_POINT('Ctrl Pts',(16.9789053705259,18.0272123578381,-5.2155134637109));
#98189=CARTESIAN_POINT('Ctrl Pts',(16.9814926820828,18.0233853992743,-5.21523216421622));
#98190=CARTESIAN_POINT('Ctrl Pts',(16.9895487919404,18.0115530536154,-5.21435795951966));
#98191=CARTESIAN_POINT('Ctrl Pts',(16.9950599823976,18.0035768755451,-5.21376228848335));
#98192=CARTESIAN_POINT('Ctrl Pts',(17.0573285124062,17.9147681396608,-5.20706090758718));
#98193=CARTESIAN_POINT('Ctrl Pts',(17.1196150883644,17.8379737651375,-5.20062764360413));
#98194=CARTESIAN_POINT('Ctrl Pts',(17.3015407181285,17.6432341265288,-5.18307319300389));
#98195=CARTESIAN_POINT('Ctrl Pts',(17.4302426694658,17.5346758175266,-5.17192748994837));
#98196=CARTESIAN_POINT('Ctrl Pts',(17.5967906923591,17.4250996310605,-5.15940133723881));
#98197=CARTESIAN_POINT('Ctrl Pts',(17.6235431133017,17.4083434034479,-5.15743871782998));
#98198=CARTESIAN_POINT('Ctrl Pts',(17.6638283057349,17.3843483036585,-5.15455519500633));
#98199=CARTESIAN_POINT('Ctrl Pts',(17.6770802748512,17.3766487280465,-5.15361788718658));
#98200=CARTESIAN_POINT('Ctrl Pts',(17.7013526899396,17.3628964935241,-5.15192118788303));
#98201=CARTESIAN_POINT('Ctrl Pts',(17.7123455761262,17.356796859432,-5.15116013442713));
#98202=CARTESIAN_POINT('Ctrl Pts',(17.7297375581182,17.3473481835301,-5.14996745028875));
#98203=CARTESIAN_POINT('Ctrl Pts',(17.7361004399357,17.3439334197088,-5.14953347939301));
#98204=CARTESIAN_POINT('Ctrl Pts',(17.7425268617009,17.340526792826,-5.14909753542998));
#98205=CARTESIAN_POINT('Ctrl Pts',(17.7425729937549,17.3405023405487,-5.14909440612938));
#98206=CARTESIAN_POINT('Ctrl Pts',(17.7426668839292,17.3404525785478,-5.14908803747501));
#98207=CARTESIAN_POINT('Ctrl Pts',(17.7427146431582,17.340427268393,-5.14908479805474));
#98208=CARTESIAN_POINT('Ctrl Pts',(17.7428118470402,17.3403757596561,-5.14907820516147));
#98209=CARTESIAN_POINT('Ctrl Pts',(17.7428612926054,17.3403495607585,-5.14907485163596));
#98210=CARTESIAN_POINT('Ctrl Pts',(17.742961930683,17.3402962424479,-5.14906802638801));
#98211=CARTESIAN_POINT('Ctrl Pts',(17.7430131240878,17.3402691227423,-5.1490645546151));
#98212=CARTESIAN_POINT('Ctrl Pts',(17.7431173215902,17.3402139295943,-5.14905748857992));
#98213=CARTESIAN_POINT('Ctrl Pts',(17.7431703265441,17.3401858558916,-5.14905389427035));
#98214=CARTESIAN_POINT('Ctrl Pts',(17.7432782132587,17.3401287203199,-5.14904657871138));
#98215=CARTESIAN_POINT('Ctrl Pts',(17.7433330958113,17.3400996582391,-5.14904285741986));
#98216=CARTESIAN_POINT('Ctrl Pts',(17.7434448062837,17.3400405102367,-5.14903528328347));
#98217=CARTESIAN_POINT('Ctrl Pts',(17.7435016349047,17.3400104241665,-5.14903143040346));
#98218=CARTESIAN_POINT('Ctrl Pts',(17.7436173084945,17.3399491912835,-5.14902358831549));
#98219=CARTESIAN_POINT('Ctrl Pts',(17.7436761541978,17.3399180443209,-5.14901959907105));
#98220=CARTESIAN_POINT('Ctrl Pts',(17.7437959355934,17.3398546514006,-5.14901147930244));
#98221=CARTESIAN_POINT('Ctrl Pts',(17.7438568718533,17.3398224053991,-5.14900734875409));
#98222=CARTESIAN_POINT('Ctrl Pts',(17.7439809105642,17.3397567748556,-5.14899894125579));
#98223=CARTESIAN_POINT('Ctrl Pts',(17.7440440136382,17.3397233902593,-5.14899466427896));
#98224=CARTESIAN_POINT('Ctrl Pts',(17.7441724649142,17.3396554416007,-5.14898595862013));
#98225=CARTESIAN_POINT('Ctrl Pts',(17.744237813652,17.3396208775503,-5.14898152991829));
#98226=CARTESIAN_POINT('Ctrl Pts',(17.7443708400812,17.3395505265439,-5.14897251517862));
#98227=CARTESIAN_POINT('Ctrl Pts',(17.744438515141,17.3395147412968,-5.14896792933687));
#98228=CARTESIAN_POINT('Ctrl Pts',(17.744565124291,17.3394478016433,-5.14895935045504));
#98229=CARTESIAN_POINT('Ctrl Pts',(17.7446240592246,17.3394166456558,-5.14895535729448));
#98230=CARTESIAN_POINT('Ctrl Pts',(17.7447516801295,17.3393491865018,-5.14894671071834));
#98231=CARTESIAN_POINT('Ctrl Pts',(17.7448203677342,17.3393128837474,-5.14894205726322));
#98232=CARTESIAN_POINT('Ctrl Pts',(17.7449690904234,17.3392342913453,-5.14893198216726));
#98233=CARTESIAN_POINT('Ctrl Pts',(17.7450491271088,17.339192002581,-5.14892656051443));
#98234=CARTESIAN_POINT('Ctrl Pts',(17.7452223978501,17.3391004662097,-5.14891482401745));
#98235=CARTESIAN_POINT('Ctrl Pts',(17.7453156336344,17.3390512200324,-5.1489085091869));
#98236=CARTESIAN_POINT('Ctrl Pts',(17.7455174426764,17.3389446458661,-5.14889484179935));
#98237=CARTESIAN_POINT('Ctrl Pts',(17.7456260177007,17.3388873201143,-5.14888748929952));
#98238=CARTESIAN_POINT('Ctrl Pts',(17.7458609758868,17.3387632923568,-5.14887157982363));
#98239=CARTESIAN_POINT('Ctrl Pts',(17.7459873605098,17.3386965938638,-5.14886302298758));
#98240=CARTESIAN_POINT('Ctrl Pts',(17.7462732875681,17.3385457351152,-5.14884366643892));
#98241=CARTESIAN_POINT('Ctrl Pts',(17.7464328340597,17.3384615824252,-5.14883286699294));
#98242=CARTESIAN_POINT('Ctrl Pts',(17.7523042951661,17.3353656433259,-5.14843549068378));
#98243=CARTESIAN_POINT('Ctrl Pts',(17.7580299971857,17.3323799607537,-5.1480498414139));
#98244=CARTESIAN_POINT('Ctrl Pts',(17.7712868462962,17.3255441073084,-5.14716118409919));
#98245=CARTESIAN_POINT('Ctrl Pts',(17.778827618023,17.32171276311,-5.14665884326033));
#98246=CARTESIAN_POINT('Ctrl Pts',(17.7991802184313,17.3115249366375,-5.14531132764273));
#98247=CARTESIAN_POINT('Ctrl Pts',(17.812033972748,17.3052528499592,-5.14446910053862));
#98248=CARTESIAN_POINT('Ctrl Pts',(17.9304952002776,17.2489278558678,-5.13678484693071));
#98249=CARTESIAN_POINT('Ctrl Pts',(18.0400203632305,17.2075667989625,-5.13025966790724));
#98250=CARTESIAN_POINT('Ctrl Pts',(18.3090877065854,17.1306900886076,-5.11494053939293));
#98251=CARTESIAN_POINT('Ctrl Pts',(18.4703869809401,17.1041692002194,-5.10633029852664));
#98252=CARTESIAN_POINT('Ctrl Pts',(18.6653452635767,17.094867431543,-5.09512044645868));
#98253=CARTESIAN_POINT('Ctrl Pts',(18.6976101780815,17.0940668302937,-5.09323781104055));
#98254=CARTESIAN_POINT('Ctrl Pts',(18.7371021607656,17.0939899493437,-5.09088633191333));
#98255=CARTESIAN_POINT('Ctrl Pts',(18.7443254861544,17.0940128581174,-5.09045430113954));
#98256=CARTESIAN_POINT('Ctrl Pts',(18.7556544325444,17.0941067703038,-5.08977348621681));
#98257=CARTESIAN_POINT('Ctrl Pts',(18.7597602832643,17.0941527529058,-5.08952607997421));
#98258=CARTESIAN_POINT('Ctrl Pts',(18.7674380386202,17.0942610789131,-5.08906215587487));
#98259=CARTESIAN_POINT('Ctrl Pts',(18.7710099280465,17.0943205185864,-5.08884580206336));
#98260=CARTESIAN_POINT('Ctrl Pts',(18.7791676957407,17.094476926914,-5.08835048726969));
#98261=CARTESIAN_POINT('Ctrl Pts',(18.7837534045061,17.0945797587744,-5.0880712025695));
#98262=CARTESIAN_POINT('Ctrl Pts',(18.7978632819704,17.0949420473855,-5.08720931090085));
#98263=CARTESIAN_POINT('Ctrl Pts',(18.8073859086107,17.0952508943102,-5.08662404703951));
#98264=CARTESIAN_POINT('Ctrl Pts',(18.9364096869498,17.1003076005152,-5.07864861266085));
#98265=CARTESIAN_POINT('Ctrl Pts',(19.0552882197228,17.1151089398747,-5.07078164892295));
#98266=CARTESIAN_POINT('Ctrl Pts',(19.2788793356495,17.1624222177002,-5.05568351915807));
#98267=CARTESIAN_POINT('Ctrl Pts',(19.3836001930243,17.1931824943587,-5.04848024951828));
#98268=CARTESIAN_POINT('Ctrl Pts',(19.5556501469808,17.2585113818391,-5.0366556210673));
#98269=CARTESIAN_POINT('Ctrl Pts',(19.6243475460686,17.2888646867418,-5.03193409089951));
#98270=CARTESIAN_POINT('Ctrl Pts',(19.708070742436,17.3313114693982,-5.02618365548227));
#98271=CARTESIAN_POINT('Ctrl Pts',(19.7247332835523,17.3400402516219,-5.02503922766813));
#98272=CARTESIAN_POINT('Ctrl Pts',(19.7488019286374,17.3530604888887,-5.02338571789685));
#98273=CARTESIAN_POINT('Ctrl Pts',(19.7563014877007,17.3571764234655,-5.02287043932883));
#98274=CARTESIAN_POINT('Ctrl Pts',(19.7694108074949,17.3644748708633,-5.02196955231988));
#98275=CARTESIAN_POINT('Ctrl Pts',(19.7750313188752,17.3676377492855,-5.02158324789162));
#98276=CARTESIAN_POINT('Ctrl Pts',(19.7859201083961,17.3738309763772,-5.02083470200891));
#98277=CARTESIAN_POINT('Ctrl Pts',(19.7911899575873,17.3768584213403,-5.02047236100222));
#98278=CARTESIAN_POINT('Ctrl Pts',(19.8037616516294,17.3841528441756,-5.01960776236391));
#98279=CARTESIAN_POINT('Ctrl Pts',(19.8110511444346,17.3884409865613,-5.01910627519593));
#98280=CARTESIAN_POINT('Ctrl Pts',(19.8372915207901,17.404089651508,-5.01730026724312));
#98281=CARTESIAN_POINT('Ctrl Pts',(19.8560903810793,17.4157032506496,-5.01600496945837));
#98282=CARTESIAN_POINT('Ctrl Pts',(20.0311433128968,17.5276718041231,-5.00391919883066));
#98283=CARTESIAN_POINT('Ctrl Pts',(20.1737328988905,17.647878196273,-4.99398659812591));
#98284=CARTESIAN_POINT('Ctrl Pts',(20.3527446000026,17.8443378473788,-4.97949718431949));
#98285=CARTESIAN_POINT('Ctrl Pts',(20.4032656567957,17.9065270474114,-4.97509387528752));
#98286=CARTESIAN_POINT('Ctrl Pts',(20.471224497983,18.0006129825604,-4.96845483110276));
#98287=CARTESIAN_POINT('Ctrl Pts',(20.4915597355171,18.030335307369,-4.96636025628068));
#98288=CARTESIAN_POINT('Ctrl Pts',(20.5151824692052,18.0668261768349,-4.96377332146848));
#98289=CARTESIAN_POINT('Ctrl Pts',(20.5192059279987,18.0731140140186,-4.96332702094746));
#98290=CARTESIAN_POINT('Ctrl Pts',(20.5254190716096,18.0829379416076,-4.96262868255573));
#98291=CARTESIAN_POINT('Ctrl Pts',(20.5276317792475,18.0864594993949,-4.9623781420078));
#98292=CARTESIAN_POINT('Ctrl Pts',(20.5317223383541,18.0930124732045,-4.96191150004868));
#98293=CARTESIAN_POINT('Ctrl Pts',(20.533602913083,18.0960421216454,-4.9616955821236));
#98294=CARTESIAN_POINT('Ctrl Pts',(20.5378451174003,18.102915102167,-4.96120536747651));
#98295=CARTESIAN_POINT('Ctrl Pts',(20.5402021108608,18.1067612204667,-4.96093077309707));
#98296=CARTESIAN_POINT('Ctrl Pts',(20.5462565717578,18.1167120774044,-4.96021969315446));
#98297=CARTESIAN_POINT('Ctrl Pts',(20.5499354570135,18.1228279768035,-4.95978204020591));
#98298=CARTESIAN_POINT('Ctrl Pts',(20.5723483664446,18.1605181182324,-4.95708172966992));
#98299=CARTESIAN_POINT('Ctrl Pts',(20.5902881255627,18.1925546551957,-4.95477276410428));
#98300=CARTESIAN_POINT('Ctrl Pts',(20.6867179057959,18.3757769882834,-4.94155887217023));
#98301=CARTESIAN_POINT('Ctrl Pts',(20.7475683513684,18.5355370038938,-4.93006551996235));
#98302=CARTESIAN_POINT('Ctrl Pts',(20.8116277076602,18.7935427779359,-4.91278865236797));
#98303=CARTESIAN_POINT('Ctrl Pts',(20.8283436779442,18.8876793428476,-4.90672137332949));
#98304=CARTESIAN_POINT('Ctrl Pts',(20.8409557532101,19.0039140454517,-4.89953959306726));
#98305=CARTESIAN_POINT('Ctrl Pts',(20.8429418773827,19.0252276953234,-4.89823491581578));
#98306=CARTESIAN_POINT('Ctrl Pts',(20.8453044512104,19.0555531311161,-4.89639535169131));
#98307=CARTESIAN_POINT('Ctrl Pts',(20.8459470553223,19.0645423126358,-4.89585214530947));
#98308=CARTESIAN_POINT('Ctrl Pts',(20.8469560512532,19.0800483917354,-4.8949186465579));
#98309=CARTESIAN_POINT('Ctrl Pts',(20.847349737989,19.0865633307368,-4.89452750254457));
#98310=CARTESIAN_POINT('Ctrl Pts',(20.8480455106944,19.0990350450933,-4.89378073458804));
#98311=CARTESIAN_POINT('Ctrl Pts',(20.8483525640714,19.1049914704365,-4.89342495845663));
#98312=CARTESIAN_POINT('Ctrl Pts',(20.8490849377019,19.1204706260673,-4.89250262626724));
#98313=CARTESIAN_POINT('Ctrl Pts',(20.8494711244829,19.1299951406741,-4.89193730086953));
#98314=CARTESIAN_POINT('Ctrl Pts',(20.8505663603021,19.1624148244431,-4.89002026407437));
#98315=CARTESIAN_POINT('Ctrl Pts',(20.850968170873,19.1853192558791,-4.88867816123748));
#98316=CARTESIAN_POINT('Ctrl Pts',(20.8512295742387,19.3848382571626,-4.87708342181251));
#98317=CARTESIAN_POINT('Ctrl Pts',(20.8293614529549,19.5607825552394,-4.86759302040801));
#98318=CARTESIAN_POINT('Ctrl Pts',(20.7646769708164,19.8155434887637,-4.85328878113131));
#98319=CARTESIAN_POINT('Ctrl Pts',(20.7383771692414,19.8977252753808,-4.84856657343219));
#98320=CARTESIAN_POINT('Ctrl Pts',(20.6935117427131,20.0131335107421,-4.84149554083877));
#98321=CARTESIAN_POINT('Ctrl Pts',(20.6789483766716,20.0478272567555,-4.83930983386104));
#98322=CARTESIAN_POINT('Ctrl Pts',(20.6603586337361,20.0890026029904,-4.836621838883));
#98323=CARTESIAN_POINT('Ctrl Pts',(20.6572108952173,20.0958762654956,-4.83616991645551));
#98324=CARTESIAN_POINT('Ctrl Pts',(20.652265838085,20.1065236707714,-4.8354646804091));
#98325=CARTESIAN_POINT('Ctrl Pts',(20.6504940099607,20.1103092791512,-4.83521291234682));
#98326=CARTESIAN_POINT('Ctrl Pts',(20.6471906365745,20.1173130199926,-4.83474516789243));
#98327=CARTESIAN_POINT('Ctrl Pts',(20.6456621714024,20.120532541435,-4.83452938247815));
#98328=CARTESIAN_POINT('Ctrl Pts',(20.6421925724225,20.1277934375356,-4.83404099175021));
#98329=CARTESIAN_POINT('Ctrl Pts',(20.6402467370215,20.1318324914427,-4.83376809826387));
#98330=CARTESIAN_POINT('Ctrl Pts',(20.6344781805794,20.1437098897379,-4.8329621038197));
#98331=CARTESIAN_POINT('Ctrl Pts',(20.6306198923733,20.1515307177956,-4.83242686573392));
#98332=CARTESIAN_POINT('Ctrl Pts',(20.6028090913762,20.2070367399427,-4.82859708356805));
#98333=CARTESIAN_POINT('Ctrl Pts',(20.577111425047,20.2538210993135,-4.82520541176137));
#98334=CARTESIAN_POINT('Ctrl Pts',(20.5406308104231,20.3146682419944,-4.82062024070629));
#98335=CARTESIAN_POINT('Ctrl Pts',(20.5313973760414,20.3296425353914,-4.81947726141034));
#98336=CARTESIAN_POINT('Ctrl Pts',(20.4960066704448,20.385467713749,-4.81516533013202));
#98337=CARTESIAN_POINT('Ctrl Pts',(20.4686350205583,20.4255299603789,-4.81196761137516));
#98338=CARTESIAN_POINT('Ctrl Pts',(20.3751395296935,20.5527580454857,-4.80153801841995));
#98339=CARTESIAN_POINT('Ctrl Pts',(20.303627718832,20.6357546801402,-4.79430521590294));
#98340=CARTESIAN_POINT('Ctrl Pts',(20.1869268522954,20.751690994199,-4.78373156033375));
#98341=CARTESIAN_POINT('Ctrl Pts',(20.1463327189766,20.7889867837565,-4.78024233014644));
#98342=CARTESIAN_POINT('Ctrl Pts',(20.0781788860306,20.8468633414559,-4.77468462939269));
#98343=CARTESIAN_POINT('Ctrl Pts',(20.0514942736566,20.8684301809681,-4.77257771781605));
#98344=CARTESIAN_POINT('Ctrl Pts',(20.0157271242064,20.8959277144478,-4.76984113922598));
#98345=CARTESIAN_POINT('Ctrl Pts',(20.0071077823162,20.9024497938846,-4.76918812982322));
#98346=CARTESIAN_POINT('Ctrl Pts',(19.9929062907476,20.9130257148125,-4.76812262418186));
#98347=CARTESIAN_POINT('Ctrl Pts',(19.9873536859432,20.9171187304674,-4.76770859846668));
#98348=CARTESIAN_POINT('Ctrl Pts',(19.9765651570821,20.9249902332771,-4.76690908268898));
#98349=CARTESIAN_POINT('Ctrl Pts',(19.9713317637717,20.9287720445831,-4.76652346627546));
#98350=CARTESIAN_POINT('Ctrl Pts',(19.9592058922682,20.9374504051987,-4.7656350491395));
#98351=CARTESIAN_POINT('Ctrl Pts',(19.9523011899901,20.9423297472438,-4.765132914467));
#98352=CARTESIAN_POINT('Ctrl Pts',(19.9336483463962,20.9553443003065,-4.76378631694572));
#98353=CARTESIAN_POINT('Ctrl Pts',(19.921846633497,20.9634022321439,-4.76294479541847));
#98354=CARTESIAN_POINT('Ctrl Pts',(19.8128225316931,21.0362338476429,-4.75526374040295));
#98355=CARTESIAN_POINT('Ctrl Pts',(19.7104705091745,21.0929796120467,-4.74874081363296));
#98356=CARTESIAN_POINT('Ctrl Pts',(19.4555786090185,21.2078722561001,-4.73343476668945));
#98357=CARTESIAN_POINT('Ctrl Pts',(19.3000126966134,21.2574096046306,-4.72483473246113));
#98358=CARTESIAN_POINT('Ctrl Pts',(19.1084258281255,21.2948788713808,-4.7136257228041));
#98359=CARTESIAN_POINT('Ctrl Pts',(19.076383470885,21.3003824802869,-4.7117296331103));
#98360=CARTESIAN_POINT('Ctrl Pts',(19.0370676313179,21.3062067735073,-4.70936318475707));
#98361=CARTESIAN_POINT('Ctrl Pts',(19.0299008343908,21.307230928516,-4.70893019429197));
#98362=CARTESIAN_POINT('Ctrl Pts',(19.0186577337376,21.3087787929985,-4.70824820021469));
#98363=CARTESIAN_POINT('Ctrl Pts',(19.0145848403025,21.3093274378569,-4.70800058240478));
#98364=CARTESIAN_POINT('Ctrl Pts',(19.0069690724334,21.3103307610446,-4.7075364795854));
#98365=CARTESIAN_POINT('Ctrl Pts',(19.0034266360555,21.3107883335948,-4.70732015994906));
#98366=CARTESIAN_POINT('Ctrl Pts',(18.9953378506481,21.3118123471456,-4.70682521104011));
#98367=CARTESIAN_POINT('Ctrl Pts',(18.9907908261307,21.3123729942122,-4.70654625989907));
#98368=CARTESIAN_POINT('Ctrl Pts',(18.9768095662562,21.3140508239046,-4.70568639707687));
#98369=CARTESIAN_POINT('Ctrl Pts',(18.9673697532037,21.3151192466088,-4.70510284624257));
#98370=CARTESIAN_POINT('Ctrl Pts',(18.8825210037021,21.3241446574914,-4.69983274965195));
#98371=CARTESIAN_POINT('Ctrl Pts',(18.806750143018,21.3281073919894,-4.69495152712518));
#98372=CARTESIAN_POINT('Ctrl Pts',(18.5460074647156,21.3277304198091,-4.67789871868947));
#98373=CARTESIAN_POINT('Ctrl Pts',(18.3618681058443,21.3032300477396,-4.66550124996916));
#98374=CARTESIAN_POINT('Ctrl Pts',(18.1318241503516,21.2412487702261,-4.65047365059779));
#98375=CARTESIAN_POINT('Ctrl Pts',(18.0809342985178,21.2254557108729,-4.64717204928174));
#98376=CARTESIAN_POINT('Ctrl Pts',(18.0188621994328,21.2035923301053,-4.64317035481114));
#98377=CARTESIAN_POINT('Ctrl Pts',(18.0070708973072,21.1993209896954,-4.64241130097009));
#98378=CARTESIAN_POINT('Ctrl Pts',(17.9884946120081,21.1924044842425,-4.64121706921076));
#98379=CARTESIAN_POINT('Ctrl Pts',(17.981684267272,21.1898287076082,-4.64077958751628));
#98380=CARTESIAN_POINT('Ctrl Pts',(17.968942133346,21.1849341479904,-4.63996165543386));
#98381=CARTESIAN_POINT('Ctrl Pts',(17.9630072727639,21.182623639504,-4.63958093314989));
#98382=CARTESIAN_POINT('Ctrl Pts',(17.9497500548354,21.1773934404949,-4.63873098376972));
#98383=CARTESIAN_POINT('Ctrl Pts',(17.9424333721073,21.1744595528021,-4.63826224048039));
#98384=CARTESIAN_POINT('Ctrl Pts',(17.9239381160256,21.1669230259619,-4.6370781191557));
#98385=CARTESIAN_POINT('Ctrl Pts',(17.9127821716643,21.1622653399452,-4.63636460666203));
#98386=CARTESIAN_POINT('Ctrl Pts',(17.8493618896023,21.135146671232,-4.63231159546641));
#98387=CARTESIAN_POINT('Ctrl Pts',(17.7979770661027,21.110680735478,-4.62904120317594));
#98388=CARTESIAN_POINT('Ctrl Pts',(17.7238770586398,21.0716616270324,-4.62431038000907));
#98389=CARTESIAN_POINT('Ctrl Pts',(17.7003571279539,21.0586992529641,-4.62280634098087));
#98390=CARTESIAN_POINT('Ctrl Pts',(17.5767140742856,20.987456731641,-4.61486880108734));
#98391=CARTESIAN_POINT('Ctrl Pts',(17.4812555646195,20.9214798729665,-4.60864386096608));
#98392=CARTESIAN_POINT('Ctrl Pts',(17.3297827366213,20.7972750668102,-4.59796498357712));
#98393=CARTESIAN_POINT('Ctrl Pts',(17.2708254705386,20.7430616847505,-4.59356323704014));
#98394=CARTESIAN_POINT('Ctrl Pts',(17.1900057768913,20.6598157038647,-4.58692631778353));
#98395=CARTESIAN_POINT('Ctrl Pts',(17.1655927649907,20.6333513989536,-4.58483220143466));
#98396=CARTESIAN_POINT('Ctrl Pts',(17.1369482569954,20.6006655889278,-4.5822457752747));
#98397=CARTESIAN_POINT('Ctrl Pts',(17.1320583328928,20.5950258705332,-4.58179950377347));
#98398=CARTESIAN_POINT('Ctrl Pts',(17.1244905668321,20.5862038690185,-4.58110120099635));
#98399=CARTESIAN_POINT('Ctrl Pts',(17.1217920484444,20.5830392913752,-4.58085066679607));
#98400=CARTESIAN_POINT('Ctrl Pts',(17.1167971345355,20.5771466275252,-4.58038403048547));
#98401=CARTESIAN_POINT('Ctrl Pts',(17.1144983004347,20.5744206835985,-4.58016811182235));
#98402=CARTESIAN_POINT('Ctrl Pts',(17.1093069070463,20.5682331057692,-4.57967788750414));
#98403=CARTESIAN_POINT('Ctrl Pts',(17.1064185330244,20.5647680440806,-4.57940328414158));
#98404=CARTESIAN_POINT('Ctrl Pts',(17.0978965100615,20.5544778343176,-4.57858763695095));
#98405=CARTESIAN_POINT('Ctrl Pts',(17.0922946412651,20.5476266606343,-4.57804438040996));
#98406=CARTESIAN_POINT('Ctrl Pts',(17.0511025773865,20.4965985139932,-4.57399795859996));
#98407=CARTESIAN_POINT('Ctrl Pts',(17.0172611142355,20.4510458272492,-4.57038509503549));
#98408=CARTESIAN_POINT('Ctrl Pts',(16.9504036025297,20.3530615930658,-4.56270240111715));
#98409=CARTESIAN_POINT('Ctrl Pts',(16.9177751785404,20.3004253513025,-4.5586247818669));
#98410=CARTESIAN_POINT('Ctrl Pts',(16.8338945767296,20.1508408274315,-4.54729667242138));
#98411=CARTESIAN_POINT('Ctrl Pts',(16.7877886618243,20.0512179998227,-4.5400480933186));
#98412=CARTESIAN_POINT('Ctrl Pts',(16.7303166545563,19.8965707557044,-4.52944127355711));
#98413=CARTESIAN_POINT('Ctrl Pts',(16.7130722627021,19.8439345326445,-4.52593476936327));
#98414=CARTESIAN_POINT('Ctrl Pts',(16.6884846754667,19.7575720160236,-4.52035278720549));
#98415=CARTESIAN_POINT('Ctrl Pts',(16.6798675391327,19.7242387002014,-4.51823844816655));
#98416=CARTESIAN_POINT('Ctrl Pts',(16.669614456483,19.6801678230864,-4.51549378176146));
#98417=CARTESIAN_POINT('Ctrl Pts',(16.6672430079269,19.6696083961618,-4.51483993910782));
#98418=CARTESIAN_POINT('Ctrl Pts',(16.6634921046976,19.6522863917352,-4.51377342232846));
#98419=CARTESIAN_POINT('Ctrl Pts',(16.6620645837058,19.6455345285478,-4.51335921312024));
#98420=CARTESIAN_POINT('Ctrl Pts',(16.659365641462,19.6324533808418,-4.51255958342342));
#98421=CARTESIAN_POINT('Ctrl Pts',(16.6580901071821,19.6261250319783,-4.51217403532362));
#98422=CARTESIAN_POINT('Ctrl Pts',(16.6552123724927,19.6115026288507,-4.51128611878298));
#98423=CARTESIAN_POINT('Ctrl Pts',(16.6536308208072,19.6032045861708,-4.51078441398248));
#98424=CARTESIAN_POINT('Ctrl Pts',(16.6495122711541,19.5808694072398,-4.50943973006159));
#98425=CARTESIAN_POINT('Ctrl Pts',(16.6470673798197,19.5668155755174,-4.50859967904288));
#98426=CARTESIAN_POINT('Ctrl Pts',(16.6261906884124,19.4391846390304,-4.50102301574524));
#98427=CARTESIAN_POINT('Ctrl Pts',(16.616903709544,19.3242992233257,-4.49459281375611));
#98428=CARTESIAN_POINT('Ctrl Pts',(16.6171578058469,19.0229639434196,-4.47808639068802));
#98429=CARTESIAN_POINT('Ctrl Pts',(16.6418924517422,18.837581013522,-4.46831880596789));
#98430=CARTESIAN_POINT('Ctrl Pts',(16.6942562459747,18.6441344240756,-4.45654184871822));
#98431=CARTESIAN_POINT('Ctrl Pts',(16.6981093691122,18.6304481264809,-4.4556994591094));
#98432=CARTESIAN_POINT('Ctrl Pts',(16.703660730018,18.6114648710771,-4.45451691988771));
#98433=CARTESIAN_POINT('Ctrl Pts',(16.7052425224818,18.6061338843476,-4.45418327483423));
#98434=CARTESIAN_POINT('Ctrl Pts',(16.70781564271,18.5975855526895,-4.45364567388351));
#98435=CARTESIAN_POINT('Ctrl Pts',(16.7087936865955,18.5943641904044,-4.453442490537));
#98436=CARTESIAN_POINT('Ctrl Pts',(16.710853077047,18.58763896931,-4.45301703896373));
#98437=CARTESIAN_POINT('Ctrl Pts',(16.7119358439217,18.5841355853084,-4.45279468524881));
#98438=CARTESIAN_POINT('Ctrl Pts',(16.7145777265398,18.5756656159272,-4.45225539030026));
#98439=CARTESIAN_POINT('Ctrl Pts',(16.7161460645308,18.5707019507145,-4.45193791291718));
#98440=CARTESIAN_POINT('Ctrl Pts',(16.7216994279354,18.5533490422127,-4.45082311741977));
#98441=CARTESIAN_POINT('Ctrl Pts',(16.7257802848631,18.5409910963517,-4.45002045320262));
#98442=CARTESIAN_POINT('Ctrl Pts',(16.7349633441649,18.5140200780063,-4.4482506304145));
#98443=CARTESIAN_POINT('Ctrl Pts',(16.7401119397152,18.4994250885034,-4.44728123638518));
#98444=CARTESIAN_POINT('Ctrl Pts',(16.7454194484637,18.4848895469342,-4.44630497835508));
#98445=CARTESIAN_POINT('Origin',(18.734,19.211,0.));
#98446=CARTESIAN_POINT('',(16.7454194503191,18.4848895418526,-3.64442446310682));
#98447=CARTESIAN_POINT('',(16.7454195180457,18.4848893563717,-3.86819359339412));
#98448=CARTESIAN_POINT('',(16.7454194503191,18.4848895418526,0.));
#98449=CARTESIAN_POINT('',(16.6170009085985,19.2129458556375,-3.91098515007265));
#98450=CARTESIAN_POINT('Ctrl Pts',(16.7454195180457,18.4848893563717,-3.86819359339412));
#98451=CARTESIAN_POINT('Ctrl Pts',(16.7340081750488,18.5161413069603,-3.8702730290524));
#98452=CARTESIAN_POINT('Ctrl Pts',(16.7233298318036,18.5476724487867,-3.87233003188037));
#98453=CARTESIAN_POINT('Ctrl Pts',(16.7086937641219,18.5945001653747,-3.87532603712808));
#98454=CARTESIAN_POINT('Ctrl Pts',(16.7041601162795,18.6095954250907,-3.87628295790638));
#98455=CARTESIAN_POINT('Ctrl Pts',(16.6975600380691,18.6324963820482,-3.87772162915976));
#98456=CARTESIAN_POINT('Ctrl Pts',(16.6953690628555,18.6402653335688,-3.87820742758997));
#98457=CARTESIAN_POINT('Ctrl Pts',(16.6915244728498,18.6542024625253,-3.87907494690955));
#98458=CARTESIAN_POINT('Ctrl Pts',(16.6898542408526,18.6603659168837,-3.87945720403082));
#98459=CARTESIAN_POINT('Ctrl Pts',(16.6863713151664,18.6734528050941,-3.88026595029803));
#98460=CARTESIAN_POINT('Ctrl Pts',(16.6845657869426,18.6803780762302,-3.88069220305471));
#98461=CARTESIAN_POINT('Ctrl Pts',(16.6809624124013,18.6944919467194,-3.8815574851934));
#98462=CARTESIAN_POINT('Ctrl Pts',(16.6791671199493,18.7016810995306,-3.88199642733997));
#98463=CARTESIAN_POINT('Ctrl Pts',(16.6747876940511,18.7196184016077,-3.88308720594793));
#98464=CARTESIAN_POINT('Ctrl Pts',(16.6722499112019,18.7303777216631,-3.88373755764843));
#98465=CARTESIAN_POINT('Ctrl Pts',(16.6345655721988,18.8959395700599,-3.89368676514654));
#98466=CARTESIAN_POINT('Ctrl Pts',(16.6168549648216,19.0541908608747,-3.90236290972166));
#98467=CARTESIAN_POINT('Ctrl Pts',(16.6170008943792,19.2129459703939,-3.91098517963697));
#98468=CARTESIAN_POINT('Ctrl Pts',(16.6170008942726,19.2129458543872,-3.91098517333644));
#98469=CARTESIAN_POINT('Ctrl Pts',(16.6171322461988,19.3558506431979,-3.91874658439979));
#98470=CARTESIAN_POINT('Ctrl Pts',(16.6317330804654,19.4983603027047,-3.9264424920887));
#98471=CARTESIAN_POINT('Ctrl Pts',(16.6625404319245,19.6478517853169,-3.93541363481339));
#98472=CARTESIAN_POINT('Ctrl Pts',(16.6645760626826,19.6573953229992,-3.9359904216043));
#98473=CARTESIAN_POINT('Ctrl Pts',(16.667882870474,19.6723895637183,-3.93690353184972));
#98474=CARTESIAN_POINT('Ctrl Pts',(16.6691098355725,19.677850007725,-3.93723750276904));
#98475=CARTESIAN_POINT('Ctrl Pts',(16.6714750781768,19.6881844490039,-3.93787242471626));
#98476=CARTESIAN_POINT('Ctrl Pts',(16.672609019639,19.6930594117202,-3.93817313382037));
#98477=CARTESIAN_POINT('Ctrl Pts',(16.6745952748942,19.7014634122482,-3.9386936798716));
#98478=CARTESIAN_POINT('Ctrl Pts',(16.6754394073226,19.7049943994331,-3.93891304719644));
#98479=CARTESIAN_POINT('Ctrl Pts',(16.6770956004237,19.7118442524171,-3.93933990619326));
#98480=CARTESIAN_POINT('Ctrl Pts',(16.6779066143187,19.7151633298341,-3.93954733136033));
#98481=CARTESIAN_POINT('Ctrl Pts',(16.6801205703334,19.7241297588524,-3.94010925993164));
#98482=CARTESIAN_POINT('Ctrl Pts',(16.6815387556165,19.7297732640509,-3.94046462903048));
#98483=CARTESIAN_POINT('Ctrl Pts',(16.6869136883268,19.7507951311197,-3.94179448535118));
#98484=CARTESIAN_POINT('Ctrl Pts',(16.6910200422985,19.7661342261252,-3.94277707608856));
#98485=CARTESIAN_POINT('Ctrl Pts',(16.7288547857979,19.9013557404675,-3.95153871836391));
#98486=CARTESIAN_POINT('Ctrl Pts',(16.7729252523116,20.0180801875818,-3.9597825681384));
#98487=CARTESIAN_POINT('Ctrl Pts',(16.8578682281151,20.1942980367638,-3.9727093888281));
#98488=CARTESIAN_POINT('Ctrl Pts',(16.8919540277664,20.256759487364,-3.97739845763347));
#98489=CARTESIAN_POINT('Ctrl Pts',(16.9780398811445,20.3971934664044,-3.98810073468003));
#98490=CARTESIAN_POINT('Ctrl Pts',(17.0322035681162,20.4736732727662,-3.99404894940884));
#98491=CARTESIAN_POINT('Ctrl Pts',(17.1051790273315,20.5634489711676,-4.00116199014754));
#98492=CARTESIAN_POINT('Ctrl Pts',(17.1193657657752,20.5803547123202,-4.00250801876747));
#98493=CARTESIAN_POINT('Ctrl Pts',(17.1384738220318,20.6024150554793,-4.00427384397666));
#98494=CARTESIAN_POINT('Ctrl Pts',(17.1431600971169,20.6077705776276,-4.00470327820077));
#98495=CARTESIAN_POINT('Ctrl Pts',(17.1524783184886,20.6183118042884,-4.00555006100294));
#98496=CARTESIAN_POINT('Ctrl Pts',(17.1571089823927,20.6234985182166,-4.00596745535447));
#98497=CARTESIAN_POINT('Ctrl Pts',(17.1660753099207,20.6334424744123,-4.00676916200921));
#98498=CARTESIAN_POINT('Ctrl Pts',(17.1704072744565,20.6382029346986,-4.00715362337432));
#98499=CARTESIAN_POINT('Ctrl Pts',(17.1803927715502,20.6490761124179,-4.0080333239212));
#98500=CARTESIAN_POINT('Ctrl Pts',(17.1860608137048,20.6551754062277,-4.00852793905558));
#98501=CARTESIAN_POINT('Ctrl Pts',(17.2012520071404,20.6713302323593,-4.00984119673477));
#98502=CARTESIAN_POINT('Ctrl Pts',(17.2108381953051,20.6813261296286,-4.01065712406613));
#98503=CARTESIAN_POINT('Ctrl Pts',(17.2870189358343,20.7592181323684,-4.01704365034278));
#98504=CARTESIAN_POINT('Ctrl Pts',(17.3580261300918,20.8226552851848,-4.02241038038099));
#98505=CARTESIAN_POINT('Ctrl Pts',(17.5136072429533,20.9438454160643,-4.03330208248319));
#98506=CARTESIAN_POINT('Ctrl Pts',(17.5985800042946,21.0006741303751,-4.03879512597839));
#98507=CARTESIAN_POINT('Ctrl Pts',(17.7562767918343,21.0903720710094,-4.04868788914964));
#98508=CARTESIAN_POINT('Ctrl Pts',(17.8273763185593,21.1256836791062,-4.0530528508949));
#98509=CARTESIAN_POINT('Ctrl Pts',(17.9331536559171,21.1710033043791,-4.05963688937138));
#98510=CARTESIAN_POINT('Ctrl Pts',(17.9663737481862,21.1842504697453,-4.06171725231584));
#98511=CARTESIAN_POINT('Ctrl Pts',(18.006866278449,21.1992204449077,-4.06428632694957));
#98512=CARTESIAN_POINT('Ctrl Pts',(18.0138348289917,21.2017551605717,-4.06472962638129));
#98513=CARTESIAN_POINT('Ctrl Pts',(18.0247533666434,21.2056618000905,-4.06542624786626));
#98514=CARTESIAN_POINT('Ctrl Pts',(18.0286944239498,21.2070587484757,-4.06567810941549));
#98515=CARTESIAN_POINT('Ctrl Pts',(18.0360021530273,21.2096247038287,-4.06614593869295));
#98516=CARTESIAN_POINT('Ctrl Pts',(18.0393676478146,21.2107968886484,-4.06636171487551));
#98517=CARTESIAN_POINT('Ctrl Pts',(18.0469717687189,21.2134238541343,-4.06684997055104));
#98518=CARTESIAN_POINT('Ctrl Pts',(18.0512120393213,21.214873669192,-4.06712273751009));
#98519=CARTESIAN_POINT('Ctrl Pts',(18.0637085721378,21.2191021610163,-4.0679280196735));
#98520=CARTESIAN_POINT('Ctrl Pts',(18.0719773023564,21.2218433129306,-4.06846266647874));
#98521=CARTESIAN_POINT('Ctrl Pts',(18.13086385684,21.2409621156783,-4.07228183069476));
#98522=CARTESIAN_POINT('Ctrl Pts',(18.1820620815793,21.2554761929898,-4.07566289750783));
#98523=CARTESIAN_POINT('Ctrl Pts',(18.376777782,21.3028290671957,-4.08861272684905));
#98524=CARTESIAN_POINT('Ctrl Pts',(18.5230453918307,21.3226005527415,-4.09849088632015));
#98525=CARTESIAN_POINT('Ctrl Pts',(18.7441911936846,21.3292698233333,-4.11289961213195));
#98526=CARTESIAN_POINT('Ctrl Pts',(18.8182691080562,21.3276179320866,-4.1176449942125));
#98527=CARTESIAN_POINT('Ctrl Pts',(18.9199296651094,21.3200038347833,-4.12402275749862));
#98528=CARTESIAN_POINT('Ctrl Pts',(18.9477017627737,21.3173709756192,-4.12575149575042));
#98529=CARTESIAN_POINT('Ctrl Pts',(18.9955496772923,21.3118787499455,-4.12870704764698));
#98530=CARTESIAN_POINT('Ctrl Pts',(19.0156508714278,21.309278481786,-4.12994170526012));
#98531=CARTESIAN_POINT('Ctrl Pts',(19.0445448247617,21.3051180828043,-4.13170687365948));
#98532=CARTESIAN_POINT('Ctrl Pts',(19.0533694336168,21.3037904342281,-4.13224469362501));
#98533=CARTESIAN_POINT('Ctrl Pts',(19.0686176354473,21.3013976725245,-4.13317184880509));
#98534=CARTESIAN_POINT('Ctrl Pts',(19.0750451444487,21.3003586580972,-4.13356200521672));
#98535=CARTESIAN_POINT('Ctrl Pts',(19.0873697610949,21.2983079814154,-4.13430888466098));
#98536=CARTESIAN_POINT('Ctrl Pts',(19.09326756453,21.2973009407909,-4.13466575028568));
#98537=CARTESIAN_POINT('Ctrl Pts',(19.108652110581,21.2946068818921,-4.13559526060995));
#98538=CARTESIAN_POINT('Ctrl Pts',(19.1181318136601,21.292880062979,-4.13616663572549));
#98539=CARTESIAN_POINT('Ctrl Pts',(19.1507198924043,21.2867136658793,-4.1381263592517));
#98540=CARTESIAN_POINT('Ctrl Pts',(19.1737663623093,21.2819534768419,-4.13950450052636));
#98541=CARTESIAN_POINT('Ctrl Pts',(19.3593649103863,21.2403804833745,-4.15055065895701));
#98542=CARTESIAN_POINT('Ctrl Pts',(19.5171301284544,21.1848745094007,-4.15955243294578));
#98543=CARTESIAN_POINT('Ctrl Pts',(19.7800786349565,21.0558148292426,-4.17547157093414));
#98544=CARTESIAN_POINT('Ctrl Pts',(19.8881758113895,20.9901827729904,-4.18235474788397));
#98545=CARTESIAN_POINT('Ctrl Pts',(19.999326516399,20.9082857073215,-4.19050259357584));
#98546=CARTESIAN_POINT('Ctrl Pts',(20.0088253297347,20.901162811534,-4.19120818886398));
#98547=CARTESIAN_POINT('Ctrl Pts',(20.0222515206398,20.8909173150772,-4.19221960688322));
#98548=CARTESIAN_POINT('Ctrl Pts',(20.0262286844835,20.8878599201322,-4.19252099295881));
#98549=CARTESIAN_POINT('Ctrl Pts',(20.0330668742742,20.8825643723634,-4.19304233376008));
#98550=CARTESIAN_POINT('Ctrl Pts',(20.0359331056542,20.8803329155817,-4.1932618149417));
#98551=CARTESIAN_POINT('Ctrl Pts',(20.0414816864101,20.8759901777714,-4.19368859086692));
#98552=CARTESIAN_POINT('Ctrl Pts',(20.0441646780786,20.8738797816756,-4.19389581772906));
#98553=CARTESIAN_POINT('Ctrl Pts',(20.0513947480816,20.8681643702373,-4.19445655064975));
#98554=CARTESIAN_POINT('Ctrl Pts',(20.0559320882067,20.864547164312,-4.19481091601459));
#98555=CARTESIAN_POINT('Ctrl Pts',(20.0727469664247,20.8510287597202,-4.19613317986286));
#98556=CARTESIAN_POINT('Ctrl Pts',(20.0849282545491,20.8410093834432,-4.19710906595625));
#98557=CARTESIAN_POINT('Ctrl Pts',(20.1966283633912,20.7470214721884,-4.20621672860228));
#98558=CARTESIAN_POINT('Ctrl Pts',(20.2883046428404,20.6541821483913,-4.21485581174275));
#98559=CARTESIAN_POINT('Ctrl Pts',(20.4727946800734,20.4292433853559,-4.23407494658443));
#98560=CARTESIAN_POINT('Ctrl Pts',(20.5602584382964,20.2937384948187,-4.24454512065337));
#98561=CARTESIAN_POINT('Ctrl Pts',(20.6409846290793,20.1305388023696,-4.25572787711943));
#98562=CARTESIAN_POINT('Ctrl Pts',(20.6501331131048,20.1113199039178,-4.25702508976319));
#98563=CARTESIAN_POINT('Ctrl Pts',(20.6627321948377,20.0837897614468,-4.25885604748058));
#98564=CARTESIAN_POINT('Ctrl Pts',(20.6664218245012,20.075589927758,-4.25939800661627));
#98565=CARTESIAN_POINT('Ctrl Pts',(20.6726978320906,20.0614012380509,-4.26033003459456));
#98566=CARTESIAN_POINT('Ctrl Pts',(20.6753089555614,20.0554235254695,-4.26072094801069));
#98567=CARTESIAN_POINT('Ctrl Pts',(20.6802562481001,20.0439533239268,-4.26146773334372));
#98568=CARTESIAN_POINT('Ctrl Pts',(20.6825968959646,20.0384628458548,-4.26182375524728));
#98569=CARTESIAN_POINT('Ctrl Pts',(20.6886244241814,20.024156607944,-4.2627477141079));
#98570=CARTESIAN_POINT('Ctrl Pts',(20.6922749185422,20.0153255911684,-4.26331441161118));
#98571=CARTESIAN_POINT('Ctrl Pts',(20.7045260611332,19.9851106327014,-4.26524118247259));
#98572=CARTESIAN_POINT('Ctrl Pts',(20.7128374213022,19.9636106235572,-4.26659151209585));
#98573=CARTESIAN_POINT('Ctrl Pts',(20.7811160665671,19.7780295815631,-4.27808140086563));
#98574=CARTESIAN_POINT('Ctrl Pts',(20.8209119827372,19.6072472051742,-4.287477931127));
#98575=CARTESIAN_POINT('Ctrl Pts',(20.8484770077298,19.3464321839502,-4.30174639421038));
#98576=CARTESIAN_POINT('Ctrl Pts',(20.852268116943,19.2588816240947,-4.30653795327146));
#98577=CARTESIAN_POINT('Ctrl Pts',(20.8499178595543,19.1334000458307,-4.31370249473699));
#98578=CARTESIAN_POINT('Ctrl Pts',(20.8481861880695,19.0954729462956,-4.31590739121543));
#98579=CARTESIAN_POINT('Ctrl Pts',(20.8448868890886,19.0500559339576,-4.31861665567595));
#98580=CARTESIAN_POINT('Ctrl Pts',(20.8442971302259,19.0424993497234,-4.31906972587955));
#98581=CARTESIAN_POINT('Ctrl Pts',(20.8433188658876,19.0307767279496,-4.31977636972615));
#98582=CARTESIAN_POINT('Ctrl Pts',(20.8429585606805,19.026608312511,-4.32002838788244));
#98583=CARTESIAN_POINT('Ctrl Pts',(20.8422684943924,19.0188915537733,-4.32049635942624));
#98584=CARTESIAN_POINT('Ctrl Pts',(20.8419421300191,19.015342964681,-4.32071212031728));
#98585=CARTESIAN_POINT('Ctrl Pts',(20.8411854477312,19.0073371894712,-4.32120015061534));
#98586=CARTESIAN_POINT('Ctrl Pts',(20.8407499494864,19.0028805607125,-4.32147270630836));
#98587=CARTESIAN_POINT('Ctrl Pts',(20.839427181919,18.9897738881274,-4.32227680003598));
#98588=CARTESIAN_POINT('Ctrl Pts',(20.83850076606,18.9811280124874,-4.32281046046641));
#98589=CARTESIAN_POINT('Ctrl Pts',(20.8315639091146,18.9199493667243,-4.32660842497082));
#98590=CARTESIAN_POINT('Ctrl Pts',(20.8236409165926,18.8676566565923,-4.32996810931569));
#98591=CARTESIAN_POINT('Ctrl Pts',(20.8132706188509,18.8130931702028,-4.33355650421712));
#98592=CARTESIAN_POINT('Ctrl Pts',(20.812766315121,18.8104669069373,-4.33372942581347));
#98593=CARTESIAN_POINT('Ctrl Pts',(20.8067039977719,18.7792160284454,-4.3357894640278));
#98594=CARTESIAN_POINT('Ctrl Pts',(20.8005602739575,18.7507090062411,-4.33769236429479));
#98595=CARTESIAN_POINT('Ctrl Pts',(20.7880170342882,18.6978360920448,-4.34125654432872));
#98596=CARTESIAN_POINT('Ctrl Pts',(20.7817674845587,18.6734393333877,-4.34291514306212));
#98597=CARTESIAN_POINT('Ctrl Pts',(20.7465826732987,18.5456179040197,-4.35166346588616));
#98598=CARTESIAN_POINT('Ctrl Pts',(20.7102414995577,18.4443876011478,-4.35878402065841));
#98599=CARTESIAN_POINT('Ctrl Pts',(20.6407861833358,18.2891647883661,-4.36977755715366));
#98600=CARTESIAN_POINT('Ctrl Pts',(20.6126715314603,18.2331410343518,-4.37376458546057));
#98601=CARTESIAN_POINT('Ctrl Pts',(20.5637633782404,18.145603349821,-4.38001455570823));
#98602=CARTESIAN_POINT('Ctrl Pts',(20.5445429626296,18.1132575403375,-4.38232895660014));
#98603=CARTESIAN_POINT('Ctrl Pts',(20.5185082980585,18.0719899184099,-4.38529025175654));
#98604=CARTESIAN_POINT('Ctrl Pts',(20.512472055782,18.0625876236719,-4.38596554896999));
#98605=CARTESIAN_POINT('Ctrl Pts',(20.5025451948745,18.0473911350403,-4.38705811331711));
#98606=CARTESIAN_POINT('Ctrl Pts',(20.4986999221598,18.0415677088988,-4.38747706243136));
#98607=CARTESIAN_POINT('Ctrl Pts',(20.4912573891632,18.030416759211,-4.38827984590693));
#98608=CARTESIAN_POINT('Ctrl Pts',(20.487664526282,18.0250864066603,-4.38866383953559));
#98609=CARTESIAN_POINT('Ctrl Pts',(20.479393289368,18.0129350281893,-4.38953982885042));
#98610=CARTESIAN_POINT('Ctrl Pts',(20.4746990886027,18.0061248624226,-4.39003121841804));
#98611=CARTESIAN_POINT('Ctrl Pts',(20.462145872562,17.9881396307921,-4.39133026000814));
#98612=CARTESIAN_POINT('Ctrl Pts',(20.4542183099843,17.9770127154291,-4.39213529052361));
#98613=CARTESIAN_POINT('Ctrl Pts',(20.3944973525776,17.894884035786,-4.39808918978787));
#98614=CARTESIAN_POINT('Ctrl Pts',(20.3384320159953,17.8270876937509,-4.40306565206366));
#98615=CARTESIAN_POINT('Ctrl Pts',(20.1821105229613,17.6603728977585,-4.41573245651121));
#98616=CARTESIAN_POINT('Ctrl Pts',(20.0759332990415,17.5676248728425,-4.42321230087426));
#98617=CARTESIAN_POINT('Ctrl Pts',(19.9155053660955,17.4534734912241,-4.43408033940308));
#98618=CARTESIAN_POINT('Ctrl Pts',(19.8683851125068,17.4226980431254,-4.4372302225456));
#98619=CARTESIAN_POINT('Ctrl Pts',(19.7953661861868,17.3790553924104,-4.44213516135802));
#98620=CARTESIAN_POINT('Ctrl Pts',(19.7703356638665,17.3647802318397,-4.44382064940801));
#98621=CARTESIAN_POINT('Ctrl Pts',(19.7388996908033,17.347692675444,-4.44595232855252));
#98622=CARTESIAN_POINT('Ctrl Pts',(19.7327600182035,17.3443945255417,-4.44636935391955));
#98623=CARTESIAN_POINT('Ctrl Pts',(19.7230269849404,17.3392278380903,-4.44703172217683));
#98624=CARTESIAN_POINT('Ctrl Pts',(19.7194442929704,17.3373391587965,-4.44727580810125));
#98625=CARTESIAN_POINT('Ctrl Pts',(19.7126825838023,17.3337993627254,-4.44773702893828));
#98626=CARTESIAN_POINT('Ctrl Pts',(19.7095047877348,17.3321460299382,-4.44795402099435));
#98627=CARTESIAN_POINT('Ctrl Pts',(19.702236843303,17.3283880978882,-4.44845082138741));
#98628=CARTESIAN_POINT('Ctrl Pts',(19.6981440273503,17.326288761559,-4.44873095591609));
#98629=CARTESIAN_POINT('Ctrl Pts',(19.6872745368124,17.3207581226272,-4.44947583675153));
#98630=CARTESIAN_POINT('Ctrl Pts',(19.6804862522674,17.3173499616336,-4.44994197293745));
#98631=CARTESIAN_POINT('Ctrl Pts',(19.6332336414111,17.2939436231039,-4.45319243317525));
#98632=CARTESIAN_POINT('Ctrl Pts',(19.5921601536008,17.2752090031939,-4.45604673137148));
#98633=CARTESIAN_POINT('Ctrl Pts',(19.5449269394488,17.2554634273718,-4.45933637506048));
#98634=CARTESIAN_POINT('Ctrl Pts',(19.5393209490136,17.2531481271879,-4.45972693248499));
#98635=CARTESIAN_POINT('Ctrl Pts',(19.387862631515,17.1913557007781,-4.4702805362724));
#98636=CARTESIAN_POINT('Ctrl Pts',(19.2358348502079,17.148316087859,-4.48087220131182));
#98637=CARTESIAN_POINT('Ctrl Pts',(18.978823441679,17.1056831256988,-4.49778517428951));
#98638=CARTESIAN_POINT('Ctrl Pts',(18.8761078637002,17.096263969277,-4.50430452206001));
#98639=CARTESIAN_POINT('Ctrl Pts',(18.7582955570908,17.0940876284215,-4.51149025665462));
#98640=CARTESIAN_POINT('Ctrl Pts',(18.7434878028228,17.0939694706699,-4.51238838544493));
#98641=CARTESIAN_POINT('Ctrl Pts',(18.7209110826764,17.0940262088427,-4.51375028545251));
#98642=CARTESIAN_POINT('Ctrl Pts',(18.7131425261603,17.0940884948827,-4.51421756807006));
#98643=CARTESIAN_POINT('Ctrl Pts',(18.699013597531,17.0942795605143,-4.51506504378658));
#98644=CARTESIAN_POINT('Ctrl Pts',(18.692653155287,17.0943942485446,-4.515445673544));
#98645=CARTESIAN_POINT('Ctrl Pts',(18.6789275077052,17.0947036354405,-4.51626520199385));
#98646=CARTESIAN_POINT('Ctrl Pts',(18.6715625897929,17.0949081177874,-4.51670378934812));
#98647=CARTESIAN_POINT('Ctrl Pts',(18.6516069464671,17.0955664481011,-4.51788911792633));
#98648=CARTESIAN_POINT('Ctrl Pts',(18.6390188360181,17.0960942534991,-4.51863353825995));
#98649=CARTESIAN_POINT('Ctrl Pts',(18.5779507759758,17.0992011129832,-4.52222980213252));
#98650=CARTESIAN_POINT('Ctrl Pts',(18.5295623668543,17.1033350158927,-4.52503267155569));
#98651=CARTESIAN_POINT('Ctrl Pts',(18.4408421035346,17.1139991568736,-4.53011151238128));
#98652=CARTESIAN_POINT('Ctrl Pts',(18.4004761606625,17.1200394114944,-4.53239919674766));
#98653=CARTESIAN_POINT('Ctrl Pts',(18.227968545886,17.1509761437617,-4.54212597035447));
#98654=CARTESIAN_POINT('Ctrl Pts',(18.098194736733,17.1872616053873,-4.54929580651753));
#98655=CARTESIAN_POINT('Ctrl Pts',(17.9142086261841,17.258164688025,-4.56013212125728));
#98656=CARTESIAN_POINT('Ctrl Pts',(17.8567132255139,17.2833095637553,-4.56362566858367));
#98657=CARTESIAN_POINT('Ctrl Pts',(17.7726608238646,17.3246085167745,-4.56901239852279));
#98658=CARTESIAN_POINT('Ctrl Pts',(17.7452021941251,17.3388556381815,-4.57081878414247));
#98659=CARTESIAN_POINT('Ctrl Pts',(17.7118128689337,17.3571193971365,-4.57308535888627));
#98660=CARTESIAN_POINT('Ctrl Pts',(17.7055759509998,17.3605719974185,-4.57351180114141));
#98661=CARTESIAN_POINT('Ctrl Pts',(17.6957925319521,17.366052590725,-4.5741857479662));
#98662=CARTESIAN_POINT('Ctrl Pts',(17.6922341938586,17.3680594979201,-4.57443192022489));
#98663=CARTESIAN_POINT('Ctrl Pts',(17.6855723082155,17.3718422686238,-4.5748948167894));
#98664=CARTESIAN_POINT('Ctrl Pts',(17.6824674432624,17.3736156996364,-4.5751113848455));
#98665=CARTESIAN_POINT('Ctrl Pts',(17.675361824098,17.3776981835285,-4.57560890163939));
#98666=CARTESIAN_POINT('Ctrl Pts',(17.6713641360052,17.3800124638946,-4.57589018517003));
#98667=CARTESIAN_POINT('Ctrl Pts',(17.6590006650335,17.3872238628522,-4.57676429174669));
#98668=CARTESIAN_POINT('Ctrl Pts',(17.6506610583673,17.3921652911963,-4.57735987974959));
#98669=CARTESIAN_POINT('Ctrl Pts',(17.5601869776788,17.4466164563788,-4.58388406151157));
#98670=CARTESIAN_POINT('Ctrl Pts',(17.4814826859414,17.5015900641994,-4.59012179372017));
#98671=CARTESIAN_POINT('Ctrl Pts',(17.308064530617,17.6411421040318,-4.604774816402));
#98672=CARTESIAN_POINT('Ctrl Pts',(17.2166673270677,17.7292942996406,-4.61320495666886));
#98673=CARTESIAN_POINT('Ctrl Pts',(17.0955488135574,17.8691493858251,-4.62512680547077));
#98674=CARTESIAN_POINT('Ctrl Pts',(17.0592295958338,17.9147629789104,-4.62882514702687));
#98675=CARTESIAN_POINT('Ctrl Pts',(17.0037574688616,17.9906615633833,-4.63467551381041));
#98676=CARTESIAN_POINT('Ctrl Pts',(16.983410959526,18.0200325898984,-4.63687121838472));
#98677=CARTESIAN_POINT('Ctrl Pts',(16.9578007194851,18.0590775099832,-4.6397042674692));
#98678=CARTESIAN_POINT('Ctrl Pts',(16.9518562191603,18.068295813163,-4.640367061492));
#98679=CARTESIAN_POINT('Ctrl Pts',(16.9422715080927,18.0834158210239,-4.64144444340265));
#98680=CARTESIAN_POINT('Ctrl Pts',(16.9385882291837,18.0892898572344,-4.64186062706176));
#98681=CARTESIAN_POINT('Ctrl Pts',(16.9315377437401,18.1006575615209,-4.64266152292562));
#98682=CARTESIAN_POINT('Ctrl Pts',(16.9281666356074,18.1061487080187,-4.64304637612918));
#98683=CARTESIAN_POINT('Ctrl Pts',(16.9204736954179,18.11880889329,-4.6439290981769));
#98684=CARTESIAN_POINT('Ctrl Pts',(16.9161691912069,18.1259883757944,-4.64442632840094));
#98685=CARTESIAN_POINT('Ctrl Pts',(16.9047787772147,18.1452445090098,-4.64575114876464));
#98686=CARTESIAN_POINT('Ctrl Pts',(16.8977698294048,18.157366371503,-4.64657594628487));
#98687=CARTESIAN_POINT('Ctrl Pts',(16.8410107609327,18.2578170897637,-4.65333770409752));
#98688=CARTESIAN_POINT('Ctrl Pts',(16.7975405588004,18.3495508932622,-4.65904108803465));
#98689=CARTESIAN_POINT('Ctrl Pts',(16.7555368256109,18.4576181896615,-4.66542626409794));
#98690=CARTESIAN_POINT('Ctrl Pts',(16.7504072005036,18.4712297160127,-4.6662248549002));
#98691=CARTESIAN_POINT('Ctrl Pts',(16.7454194645813,18.4848895027932,-4.66702131702538));
#98692=CARTESIAN_POINT('',(16.6170000029932,19.2108919596605,-3.68920542541543));
#98693=CARTESIAN_POINT('Ctrl Pts',(16.7454194484637,18.4848895469342,-4.44630497835508));
#98694=CARTESIAN_POINT('Ctrl Pts',(16.7620249656267,18.4394124320693,-4.44325057557546));
#98695=CARTESIAN_POINT('Ctrl Pts',(16.7801860430651,18.3945172195639,-4.44012925146104));
#98696=CARTESIAN_POINT('Ctrl Pts',(16.8760920383706,18.1790053847587,-4.42474708365561));
#98697=CARTESIAN_POINT('Ctrl Pts',(16.9747456858919,18.0185744946775,-4.41214842973718));
#98698=CARTESIAN_POINT('Ctrl Pts',(17.1286539258257,17.8298074633418,-4.39674509051351));
#98699=CARTESIAN_POINT('Ctrl Pts',(17.1657754124566,17.7877988861886,-4.39326452647925));
#98700=CARTESIAN_POINT('Ctrl Pts',(17.2128424242685,17.7386164181891,-4.38912059089443));
#98701=CARTESIAN_POINT('Ctrl Pts',(17.2212358030051,17.7299941675128,-4.38839135421871));
#98702=CARTESIAN_POINT('Ctrl Pts',(17.2352366312937,17.7158547796949,-4.38719075325615));
#98703=CARTESIAN_POINT('Ctrl Pts',(17.2408020484296,17.7102965831959,-4.38671755965911));
#98704=CARTESIAN_POINT('Ctrl Pts',(17.2509287316874,17.700295145678,-4.3858637871393));
#98705=CARTESIAN_POINT('Ctrl Pts',(17.2554792919944,17.6958412422664,-4.38548273971838));
#98706=CARTESIAN_POINT('Ctrl Pts',(17.2652853260212,17.6863297393664,-4.38466714671523));
#98707=CARTESIAN_POINT('Ctrl Pts',(17.2705469932532,17.6812786213472,-4.38423288667315));
#98708=CARTESIAN_POINT('Ctrl Pts',(17.2849676783071,17.6675774925376,-4.38305175984437));
#98709=CARTESIAN_POINT('Ctrl Pts',(17.2941780629657,17.6589817959136,-4.38230723793986));
#98710=CARTESIAN_POINT('Ctrl Pts',(17.3433130964687,17.6139398315135,-4.37838616825592));
#98711=CARTESIAN_POINT('Ctrl Pts',(17.384548059278,17.5789487052456,-4.37527146450083));
#98712=CARTESIAN_POINT('Ctrl Pts',(17.5775417212019,17.4274997805049,-4.36137520083457));
#98713=CARTESIAN_POINT('Ctrl Pts',(17.7432942790343,17.3303710424829,-4.3513511588659));
#98714=CARTESIAN_POINT('Ctrl Pts',(17.9351029415774,17.2504576574925,-4.33980018026887));
#98715=CARTESIAN_POINT('Ctrl Pts',(17.9504506366743,17.2442734908208,-4.33887557450857));
#98716=CARTESIAN_POINT('Ctrl Pts',(18.0154339535036,17.2189706350912,-4.33495322615693));
#98717=CARTESIAN_POINT('Ctrl Pts',(18.0657043652678,17.201547814133,-4.3319007851306));
#98718=CARTESIAN_POINT('Ctrl Pts',(18.1249045926734,17.1834971859942,-4.32822792186033));
#98719=CARTESIAN_POINT('Ctrl Pts',(18.1332520143669,17.1810081951184,-4.32770825126156));
#98720=CARTESIAN_POINT('Ctrl Pts',(18.1459165545096,17.1773169022518,-4.32691678638023));
#98721=CARTESIAN_POINT('Ctrl Pts',(18.1502226383851,17.1760766421942,-4.32664715077164));
#98722=CARTESIAN_POINT('Ctrl Pts',(18.1579603176427,17.1738745779117,-4.32616163556875));
#98723=CARTESIAN_POINT('Ctrl Pts',(18.1613904299153,17.1729077594677,-4.32594605136858));
#98724=CARTESIAN_POINT('Ctrl Pts',(18.1688504977366,17.1708253690799,-4.32547639907788));
#98725=CARTESIAN_POINT('Ctrl Pts',(18.1728812693288,17.1697130887721,-4.3252221491604));
#98726=CARTESIAN_POINT('Ctrl Pts',(18.1842164963819,17.1666212745397,-4.32450582909725));
#98727=CARTESIAN_POINT('Ctrl Pts',(18.1915282239849,17.1646689802918,-4.32404222692731));
#98728=CARTESIAN_POINT('Ctrl Pts',(18.2353814299639,17.1532113429672,-4.32125312542023));
#98729=CARTESIAN_POINT('Ctrl Pts',(18.2721590049323,17.1446464187521,-4.31887852361217));
#98730=CARTESIAN_POINT('Ctrl Pts',(18.3941221173814,17.1196615511405,-4.31093048639852));
#98731=CARTESIAN_POINT('Ctrl Pts',(18.4800854786699,17.1074936442186,-4.30521497620494));
#98732=CARTESIAN_POINT('Ctrl Pts',(18.7418157171605,17.0867258582925,-4.28786815532137));
#98733=CARTESIAN_POINT('Ctrl Pts',(18.9181716279832,17.0947046239889,-4.27632337620133));
#98734=CARTESIAN_POINT('Ctrl Pts',(19.1141662431538,17.1282878346254,-4.26408405820796));
#98735=CARTESIAN_POINT('Ctrl Pts',(19.1367362449317,17.1325342392916,-4.26268222168468));
#98736=CARTESIAN_POINT('Ctrl Pts',(19.1685805826328,17.1390637654035,-4.26071444352681));
#98737=CARTESIAN_POINT('Ctrl Pts',(19.1779148116963,17.1410435541648,-4.26013887850158));
#98738=CARTESIAN_POINT('Ctrl Pts',(19.1930631128783,17.1443636867127,-4.2592067284491));
#98739=CARTESIAN_POINT('Ctrl Pts',(19.1988853884152,17.1456656034013,-4.25884891751254));
#98740=CARTESIAN_POINT('Ctrl Pts',(19.2110640073146,17.1484429677316,-4.25810141360815));
#98741=CARTESIAN_POINT('Ctrl Pts',(19.2174191975524,17.1499232281783,-4.25771187956592));
#98742=CARTESIAN_POINT('Ctrl Pts',(19.2325268223556,17.1535158391959,-4.25678710590187));
#98743=CARTESIAN_POINT('Ctrl Pts',(19.2412728705851,17.1556546997766,-4.25625272542227));
#98744=CARTESIAN_POINT('Ctrl Pts',(19.2707158970647,17.1630544256209,-4.25445689210552));
#98745=CARTESIAN_POINT('Ctrl Pts',(19.2913472681243,17.1685727426381,-4.2532037504682));
#98746=CARTESIAN_POINT('Ctrl Pts',(19.4033610469702,17.2003570717855,-4.24642344852745));
#98747=CARTESIAN_POINT('Ctrl Pts',(19.4929830863256,17.2324457495615,-4.24109060896725));
#98748=CARTESIAN_POINT('Ctrl Pts',(19.7363290492884,17.3385540063705,-4.22648541345346));
#98749=CARTESIAN_POINT('Ctrl Pts',(19.88369455115,17.4252486076997,-4.21752248432758));
#98750=CARTESIAN_POINT('Ctrl Pts',(20.0485716662607,17.5511900349048,-4.20567642017467));
#98751=CARTESIAN_POINT('Ctrl Pts',(20.0774798263531,17.5745008812832,-4.20352010454318));
#98752=CARTESIAN_POINT('Ctrl Pts',(20.1112138078694,17.6031995039757,-4.2008871101654));
#98753=CARTESIAN_POINT('Ctrl Pts',(20.1166458737412,17.6078684732283,-4.20045940457657));
#98754=CARTESIAN_POINT('Ctrl Pts',(20.1254659337047,17.615527664116,-4.19975863979839));
#98755=CARTESIAN_POINT('Ctrl Pts',(20.1288682832835,17.6185013687127,-4.19948677509155));
#98756=CARTESIAN_POINT('Ctrl Pts',(20.1349389071423,17.6238415647845,-4.19899887720807));
#98757=CARTESIAN_POINT('Ctrl Pts',(20.1376107447251,17.6262039257234,-4.19878315211469));
#98758=CARTESIAN_POINT('Ctrl Pts',(20.1433811713299,17.6313320083437,-4.19831508772185));
#98759=CARTESIAN_POINT('Ctrl Pts',(20.1464775521571,17.6341000621692,-4.19806257687245));
#98760=CARTESIAN_POINT('Ctrl Pts',(20.155096855643,17.6418511668158,-4.19735594333158));
#98761=CARTESIAN_POINT('Ctrl Pts',(20.160601626241,17.6468541851759,-4.19690035309468));
#98762=CARTESIAN_POINT('Ctrl Pts',(20.1922823378131,17.6759536021983,-4.19425401833392));
#98763=CARTESIAN_POINT('Ctrl Pts',(20.2178722324698,17.7006763021852,-4.19201972357592));
#98764=CARTESIAN_POINT('Ctrl Pts',(20.2978737025376,17.7819629654504,-4.18475230362379));
#98765=CARTESIAN_POINT('Ctrl Pts',(20.3497657938878,17.8409098421037,-4.17960085634584));
#98766=CARTESIAN_POINT('Ctrl Pts',(20.5145155982759,18.0504681821764,-4.16200639681164));
#98767=CARTESIAN_POINT('Ctrl Pts',(20.6105696632863,18.2132099644645,-4.14960154753646));
#98768=CARTESIAN_POINT('Ctrl Pts',(20.6923613731792,18.4066450944228,-4.13668937275581));
#98769=CARTESIAN_POINT('Ctrl Pts',(20.7005562747561,18.4268937849937,-4.13535698179561));
#98770=CARTESIAN_POINT('Ctrl Pts',(20.7114731241142,18.4551164841424,-4.13352578843577));
#98771=CARTESIAN_POINT('Ctrl Pts',(20.7144628545145,18.4629848054826,-4.13301801878129));
#98772=CARTESIAN_POINT('Ctrl Pts',(20.7195266870702,18.476554915179,-4.13214696532309));
#98773=CARTESIAN_POINT('Ctrl Pts',(20.7216233343735,18.482248128969,-4.13178293017799));
#98774=CARTESIAN_POINT('Ctrl Pts',(20.7259001319133,18.4940170641886,-4.13103327082618));
#98775=CARTESIAN_POINT('Ctrl Pts',(20.7280770281984,18.5000939071883,-4.13064775833854));
#98776=CARTESIAN_POINT('Ctrl Pts',(20.733086308776,18.5142814531294,-4.12975131614767));
#98777=CARTESIAN_POINT('Ctrl Pts',(20.7358971970614,18.522399666566,-4.12924110468477));
#98778=CARTESIAN_POINT('Ctrl Pts',(20.7447680635358,18.548533347581,-4.12760727508147));
#98779=CARTESIAN_POINT('Ctrl Pts',(20.7506349745345,18.5666137142693,-4.1264900305016));
#98780=CARTESIAN_POINT('Ctrl Pts',(20.7788920163266,18.6578631287926,-4.120913651131));
#98781=CARTESIAN_POINT('Ctrl Pts',(20.7975483763162,18.732132953823,-4.11657752005548));
#98782=CARTESIAN_POINT('Ctrl Pts',(20.8330984319958,18.9151157095607,-4.10621809926495));
#98783=CARTESIAN_POINT('Ctrl Pts',(20.8456247103672,19.0244426514256,-4.1003042143357));
#98784=CARTESIAN_POINT('Ctrl Pts',(20.8521450700533,19.20417631853,-4.09050918107038));
#98785=CARTESIAN_POINT('Ctrl Pts',(20.8512132815947,19.2741813194231,-4.08667312437598));
#98786=CARTESIAN_POINT('Ctrl Pts',(20.8437778763291,19.3922927393893,-4.07998901581291));
#98787=CARTESIAN_POINT('Ctrl Pts',(20.8390840555645,19.4404560576827,-4.07720291383589));
#98788=CARTESIAN_POINT('Ctrl Pts',(20.8317294531977,19.4960968759273,-4.07387081254261));
#98789=CARTESIAN_POINT('Ctrl Pts',(20.830671497921,19.5037758752394,-4.07340842477671));
#98790=CARTESIAN_POINT('Ctrl Pts',(20.828912092067,19.5160473874809,-4.07266521383919));
#98791=CARTESIAN_POINT('Ctrl Pts',(20.8282376436474,19.5206437841873,-4.07238587442976));
#98792=CARTESIAN_POINT('Ctrl Pts',(20.8270154825512,19.5287861923158,-4.0718892636066));
#98793=CARTESIAN_POINT('Ctrl Pts',(20.8264738777351,19.532333074951,-4.07167234005033));
#98794=CARTESIAN_POINT('Ctrl Pts',(20.8253058135114,19.5398543477503,-4.07121105941479));
#98795=CARTESIAN_POINT('Ctrl Pts',(20.8246770502732,19.543828271783,-4.07096657960802));
#98796=CARTESIAN_POINT('Ctrl Pts',(20.8229472865175,19.554562436088,-4.07030419714244));
#98797=CARTESIAN_POINT('Ctrl Pts',(20.8218248108308,19.5613190969023,-4.06988510580349));
#98798=CARTESIAN_POINT('Ctrl Pts',(20.8160616767009,19.5949980782503,-4.06778578079572));
#98799=CARTESIAN_POINT('Ctrl Pts',(20.810933198114,19.6218329052306,-4.0660800940292));
#98800=CARTESIAN_POINT('Ctrl Pts',(20.7945516614194,19.6993786360622,-4.06106963058264));
#98801=CARTESIAN_POINT('Ctrl Pts',(20.7819501487824,19.7497822407039,-4.05771129351724));
#98802=CARTESIAN_POINT('Ctrl Pts',(20.728915616357,19.932986079694,-4.04524289270576));
#98803=CARTESIAN_POINT('Ctrl Pts',(20.6773010160004,20.0621977215373,-4.03596170781975));
#98804=CARTESIAN_POINT('Ctrl Pts',(20.5694994528494,20.2701183092783,-4.02080213828596));
#98805=CARTESIAN_POINT('Ctrl Pts',(20.5199100817507,20.3517538662043,-4.01477697040225));
#98806=CARTESIAN_POINT('Ctrl Pts',(20.45699767181,20.441105702491,-4.00810821764091));
#98807=CARTESIAN_POINT('Ctrl Pts',(20.4489088808851,20.4523575475894,-4.00726685070598));
#98808=CARTESIAN_POINT('Ctrl Pts',(20.4357824552206,20.4702437568369,-4.00592662479235));
#98809=CARTESIAN_POINT('Ctrl Pts',(20.4308152354769,20.4769290753352,-4.00542505943387));
#98810=CARTESIAN_POINT('Ctrl Pts',(20.4219393547239,20.4887289094744,-4.00453859377909));
#98811=CARTESIAN_POINT('Ctrl Pts',(20.4180466000976,20.4938552067366,-4.00415307848769));
#98812=CARTESIAN_POINT('Ctrl Pts',(20.4099010132332,20.5044810098667,-4.0033531060857));
#98813=CARTESIAN_POINT('Ctrl Pts',(20.4056443449131,20.5099774882321,-4.00293880665209));
#98814=CARTESIAN_POINT('Ctrl Pts',(20.3945498387777,20.5241585614896,-4.0018685547175));
#98815=CARTESIAN_POINT('Ctrl Pts',(20.3876708670395,20.5328108205002,-4.00121424552423));
#98816=CARTESIAN_POINT('Ctrl Pts',(20.3577877663349,20.5697988685039,-3.99841088458837));
#98817=CARTESIAN_POINT('Ctrl Pts',(20.3341199286135,20.5975920540963,-3.99628870474889));
#98818=CARTESIAN_POINT('Ctrl Pts',(20.2696433376916,20.6694561365765,-3.99074445329885));
#98819=CARTESIAN_POINT('Ctrl Pts',(20.227657142821,20.7124272886774,-3.98737030902173));
#98820=CARTESIAN_POINT('Ctrl Pts',(20.0622964968734,20.8678549193019,-3.97479975202564));
#98821=CARTESIAN_POINT('Ctrl Pts',(19.927618280039,20.9673620826633,-3.96601316266627));
#98822=CARTESIAN_POINT('Ctrl Pts',(19.7353992324203,21.0769713672813,-3.95357996357705));
#98823=CARTESIAN_POINT('Ctrl Pts',(19.6871154652365,21.1020894746051,-3.9504601531847));
#98824=CARTESIAN_POINT('Ctrl Pts',(19.6300004002602,21.1290586639559,-3.94671222584627));
#98825=CARTESIAN_POINT('Ctrl Pts',(19.6220551633231,21.1327501857783,-3.94618958994098));
#98826=CARTESIAN_POINT('Ctrl Pts',(19.6100019587384,21.138259646859,-3.94539448762135));
#98827=CARTESIAN_POINT('Ctrl Pts',(19.6059106294689,21.1401140535201,-3.94512420967365));
#98828=CARTESIAN_POINT('Ctrl Pts',(19.5985621659807,21.1434166132796,-3.94463801075401));
#98829=CARTESIAN_POINT('Ctrl Pts',(19.5953072507833,21.1448695730536,-3.9444223888364));
#98830=CARTESIAN_POINT('Ctrl Pts',(19.5882336157606,21.1480057679612,-3.94395320716877));
#98831=CARTESIAN_POINT('Ctrl Pts',(19.5844136345005,21.1496859118929,-3.94369946860464));
#98832=CARTESIAN_POINT('Ctrl Pts',(19.5736871819762,21.1543659293477,-3.94298600125315));
#98833=CARTESIAN_POINT('Ctrl Pts',(19.5667697172808,21.1573402305329,-3.94252475956089));
#98834=CARTESIAN_POINT('Ctrl Pts',(19.5256767420092,21.1747498014775,-3.93977873585652));
#98835=CARTESIAN_POINT('Ctrl Pts',(19.4911446417989,21.1883206491528,-3.93744656293871));
#98836=CARTESIAN_POINT('Ctrl Pts',(19.3771474976469,21.2296967447004,-3.92970862206491));
#98837=CARTESIAN_POINT('Ctrl Pts',(19.2963809359632,21.2536700894198,-3.92416829951151));
#98838=CARTESIAN_POINT('Ctrl Pts',(19.0395605479547,21.31351114945,-3.90674952948735));
#98839=CARTESIAN_POINT('Ctrl Pts',(18.8602027372249,21.3318532059096,-3.8949453656144));
#98840=CARTESIAN_POINT('Ctrl Pts',(18.6579996993966,21.3267567728553,-3.88249941011351));
#98841=CARTESIAN_POINT('Ctrl Pts',(18.6353504317566,21.325821763873,-3.88111599049576));
#98842=CARTESIAN_POINT('Ctrl Pts',(18.6032427359117,21.3239793300108,-3.87916934217481));
#98843=CARTESIAN_POINT('Ctrl Pts',(18.5937692830264,21.3233717622078,-3.87859676825141));
#98844=CARTESIAN_POINT('Ctrl Pts',(18.5783578798885,21.3222792373476,-3.87766813725326));
#98845=CARTESIAN_POINT('Ctrl Pts',(18.5724174028572,21.3218329050486,-3.87731087257365));
#98846=CARTESIAN_POINT('Ctrl Pts',(18.5599662039822,21.3208445249716,-3.87656345565097));
#98847=CARTESIAN_POINT('Ctrl Pts',(18.553455939165,21.3202974008616,-3.87617346696461));
#98848=CARTESIAN_POINT('Ctrl Pts',(18.5379367816161,21.3189207907336,-3.87524568980076));
#98849=CARTESIAN_POINT('Ctrl Pts',(18.5289304209558,21.3180636718499,-3.87470877550605));
#98850=CARTESIAN_POINT('Ctrl Pts',(18.4984286699317,21.3149634549216,-3.87289532596846));
#98851=CARTESIAN_POINT('Ctrl Pts',(18.4769617861304,21.3124488998514,-3.87162732920009));
#98852=CARTESIAN_POINT('Ctrl Pts',(18.3591357262543,21.2968145935176,-3.86470776720767));
#98853=CARTESIAN_POINT('Ctrl Pts',(18.263724968455,21.2773954969086,-3.8592599985852));
#98854=CARTESIAN_POINT('Ctrl Pts',(18.0202879377967,21.2101056222789,-3.84537888154959));
#98855=CARTESIAN_POINT('Ctrl Pts',(17.8756193290227,21.1523869789401,-3.83716565171484));
#98856=CARTESIAN_POINT('Ctrl Pts',(17.6957476336115,21.0565557328634,-3.82565615901801));
#98857=CARTESIAN_POINT('Ctrl Pts',(17.6537198992097,21.0322737453101,-3.82286191755898));
#98858=CARTESIAN_POINT('Ctrl Pts',(17.6054139183755,21.0021040126113,-3.81948067198155));
#98859=CARTESIAN_POINT('Ctrl Pts',(17.5982876030213,20.9975938188672,-3.81897739486701));
#98860=CARTESIAN_POINT('Ctrl Pts',(17.5875083648538,20.9906811636917,-3.81820903904099));
#98861=CARTESIAN_POINT('Ctrl Pts',(17.5838355254244,20.9883097069714,-3.8179459734449));
#98862=CARTESIAN_POINT('Ctrl Pts',(17.5773397178244,20.984086965744,-3.81747842453225));
#98863=CARTESIAN_POINT('Ctrl Pts',(17.5745138062785,20.9822402894084,-3.81727425011606));
#98864=CARTESIAN_POINT('Ctrl Pts',(17.5716708396979,20.9803727486796,-3.81706805653115));
#98865=CARTESIAN_POINT('Ctrl Pts',(17.5716493924919,20.980358659482,-3.81706650097145));
#98866=CARTESIAN_POINT('Ctrl Pts',(17.5716069177775,20.9803307556911,-3.81706342020347));
#98867=CARTESIAN_POINT('Ctrl Pts',(17.5715858903259,20.9803169411565,-3.81706189500105));
#98868=CARTESIAN_POINT('Ctrl Pts',(17.5715442301954,20.9802895703806,-3.81705887314492));
#98869=CARTESIAN_POINT('Ctrl Pts',(17.5715235974604,20.9802760141222,-3.81705737648873));
#98870=CARTESIAN_POINT('Ctrl Pts',(17.5714827032911,20.9802491445358,-3.8170544100272));
#98871=CARTESIAN_POINT('Ctrl Pts',(17.5714624419069,20.980235831259,-3.81705294022697));
#98872=CARTESIAN_POINT('Ctrl Pts',(17.5714222691765,20.9802094337192,-3.81705002593934));
#98873=CARTESIAN_POINT('Ctrl Pts',(17.5714023576909,20.9801963493816,-3.81704858144319));
#98874=CARTESIAN_POINT('Ctrl Pts',(17.5713628642758,20.9801703963112,-3.81704571628188));
#98875=CARTESIAN_POINT('Ctrl Pts',(17.5713432824778,20.9801575276808,-3.81704429562755));
#98876=CARTESIAN_POINT('Ctrl Pts',(17.5713044297303,20.9801319937775,-3.81704147679644));
#98877=CARTESIAN_POINT('Ctrl Pts',(17.5712851588656,20.980119328575,-3.817040078627));
#98878=CARTESIAN_POINT('Ctrl Pts',(17.5712469104831,20.9800941900686,-3.81703730349935));
#98879=CARTESIAN_POINT('Ctrl Pts',(17.5712279329782,20.9800817167869,-3.81703592654319));
#98880=CARTESIAN_POINT('Ctrl Pts',(17.5711902553968,20.9800569516996,-3.81703319269038));
#98881=CARTESIAN_POINT('Ctrl Pts',(17.5711715550792,20.9800446597483,-3.81703183577725));
#98882=CARTESIAN_POINT('Ctrl Pts',(17.5711344159396,20.9800202468866,-3.81702914085743));
#98883=CARTESIAN_POINT('Ctrl Pts',(17.5711159772758,20.980008126092,-3.81702780286318));
#98884=CARTESIAN_POINT('Ctrl Pts',(17.5710793469747,20.9799840460674,-3.81702514473397));
#98885=CARTESIAN_POINT('Ctrl Pts',(17.5710611554,20.9799720868896,-3.81702382460445));
#98886=CARTESIAN_POINT('Ctrl Pts',(17.5710250065701,20.9799483217773,-3.81702120128523));
#98887=CARTESIAN_POINT('Ctrl Pts',(17.5710070488909,20.9799365155744,-3.81701989806558));
#98888=CARTESIAN_POINT('Ctrl Pts',(17.5709713539729,20.9799130473178,-3.81701730756133));
#98889=CARTESIAN_POINT('Ctrl Pts',(17.5709536169827,20.979901385437,-3.81701602029553));
#98890=CARTESIAN_POINT('Ctrl Pts',(17.5709183522129,20.9798781984695,-3.81701346088627));
#98891=CARTESIAN_POINT('Ctrl Pts',(17.5709008241268,20.9798666731902,-3.81701218872128));
#98892=CARTESIAN_POINT('Ctrl Pts',(17.5708659653909,20.9798437517102,-3.81700965866119));
#98893=CARTESIAN_POINT('Ctrl Pts',(17.5708486347621,20.9798323555316,-3.8170084007683));
#98894=CARTESIAN_POINT('Ctrl Pts',(17.5708141596542,20.9798096848559,-3.8170058984352));
#98895=CARTESIAN_POINT('Ctrl Pts',(17.5707970154369,20.9797984105388,-3.81700465401463));
#98896=CARTESIAN_POINT('Ctrl Pts',(17.5707629036413,20.9797759773548,-3.81700217793771));
#98897=CARTESIAN_POINT('Ctrl Pts',(17.5707459358579,20.9797648183603,-3.81700094626705));
#98898=CARTESIAN_POINT('Ctrl Pts',(17.5707121667196,20.9797426091284,-3.81699849495055));
#98899=CARTESIAN_POINT('Ctrl Pts',(17.5706953655069,20.9797315589912,-3.81699727531558));
#98900=CARTESIAN_POINT('Ctrl Pts',(17.5706619203325,20.9797095614578,-3.81699484740584));
#98901=CARTESIAN_POINT('Ctrl Pts',(17.5706452764654,20.9796986141304,-3.81699363913847));
#98902=CARTESIAN_POINT('Ctrl Pts',(17.5706121369901,20.9796768163209,-3.81699123331268));
#98903=CARTESIAN_POINT('Ctrl Pts',(17.5705956415121,20.9796659659306,-3.81699003576421));
#98904=CARTESIAN_POINT('Ctrl Pts',(17.5705627911449,20.979644356968,-3.8169876508208));
#98905=CARTESIAN_POINT('Ctrl Pts',(17.5705464359826,20.9796335982216,-3.8169864634065));
#98906=CARTESIAN_POINT('Ctrl Pts',(17.5705138573104,20.979612166685,-3.816984098084));
#98907=CARTESIAN_POINT('Ctrl Pts',(17.5704976341029,20.9796014940989,-3.81698292019817));
#98908=CARTESIAN_POINT('Ctrl Pts',(17.5669721938763,20.9772821813513,-3.81672695004972));
#98909=CARTESIAN_POINT('Ctrl Pts',(17.5634698905235,20.9749631250476,-3.81647145549824));
#98910=CARTESIAN_POINT('Ctrl Pts',(17.5533724216286,20.968233754693,-3.81573140954562));
#98911=CARTESIAN_POINT('Ctrl Pts',(17.5467952015199,20.9637968248909,-3.8152451176077));
#98912=CARTESIAN_POINT('Ctrl Pts',(17.5031594114367,20.9340022629206,-3.81199132894857));
#98913=CARTESIAN_POINT('Ctrl Pts',(17.4668935509768,20.9075099297967,-3.80915427221634));
#98914=CARTESIAN_POINT('Ctrl Pts',(17.3375093174381,20.8065307137936,-3.79861576237224));
#98915=CARTESIAN_POINT('Ctrl Pts',(17.2498869211711,20.7253682148947,-3.79066785675721));
#98916=CARTESIAN_POINT('Ctrl Pts',(17.0706999415654,20.528822475985,-3.77314902005174));
#98917=CARTESIAN_POINT('Ctrl Pts',(16.9833620424435,20.4103768616343,-3.7636919082579));
#98918=CARTESIAN_POINT('Ctrl Pts',(16.9017534031063,20.271549022565,-3.75385956517648));
#98919=CARTESIAN_POINT('Ctrl Pts',(16.8946602014013,20.2591989038074,-3.75299453283563));
#98920=CARTESIAN_POINT('Ctrl Pts',(16.8835622998991,20.2394165316241,-3.75162399002801));
#98921=CARTESIAN_POINT('Ctrl Pts',(16.8794765893048,20.2320304436593,-3.75111557640561));
#98922=CARTESIAN_POINT('Ctrl Pts',(16.8723447231156,20.2189535157891,-3.75022118303641));
#98923=CARTESIAN_POINT('Ctrl Pts',(16.8692802351493,20.213272847058,-3.74983455170444));
#98924=CARTESIAN_POINT('Ctrl Pts',(16.8629918195743,20.2014872791555,-3.74903629270852));
#98925=CARTESIAN_POINT('Ctrl Pts',(16.8597716754549,20.195380439971,-3.74862480281219));
#98926=CARTESIAN_POINT('Ctrl Pts',(16.8515748731151,20.1796495893643,-3.74757024385822));
#98927=CARTESIAN_POINT('Ctrl Pts',(16.846642079434,20.1700028527513,-3.74692872674609));
#98928=CARTESIAN_POINT('Ctrl Pts',(16.8262991591984,20.129454598265,-3.74425336103823));
#98929=CARTESIAN_POINT('Ctrl Pts',(16.8115716784683,20.0982152478476,-3.74224337432153));
#98930=CARTESIAN_POINT('Ctrl Pts',(16.7751408963554,20.0157681730833,-3.7370586361944));
#98931=CARTESIAN_POINT('Ctrl Pts',(16.7546789088779,19.9640401575799,-3.73392409547238));
#98932=CARTESIAN_POINT('Ctrl Pts',(16.7027485980965,19.8159559085773,-3.72520196171289));
#98933=CARTESIAN_POINT('Ctrl Pts',(16.676126623379,19.7180621230921,-3.71973258579423));
#98934=CARTESIAN_POINT('Ctrl Pts',(16.6333093437204,19.4998588572485,-3.70764141857151));
#98935=CARTESIAN_POINT('Ctrl Pts',(16.620235005192,19.3793155006776,-3.70102399953171));
#98936=CARTESIAN_POINT('Ctrl Pts',(16.6172719227627,19.2468288732992,-3.69321427594124));
#98937=CARTESIAN_POINT('Ctrl Pts',(16.6171084252312,19.2353209518181,-3.69253143385636));
#98938=CARTESIAN_POINT('Ctrl Pts',(16.6170172121696,19.2202502263473,-3.69163065589168));
#98939=CARTESIAN_POINT('Ctrl Pts',(16.6170046437703,19.2166878770101,-3.6914172562726));
#98940=CARTESIAN_POINT('Ctrl Pts',(16.6170002821712,19.2123438082719,-3.69115642739275));
#98941=CARTESIAN_POINT('Ctrl Pts',(16.6169999302848,19.2115620757113,-3.69110946645803));
#98942=CARTESIAN_POINT('Ctrl Pts',(16.6170000113955,19.2107803447323,-3.69106248172613));
#98943=CARTESIAN_POINT('Ctrl Pts',(16.6170000023184,19.210900923828,-3.6890562790225));
#98944=CARTESIAN_POINT('Ctrl Pts',(16.6170002492315,19.2056250329456,-3.68873698393553));
#98945=CARTESIAN_POINT('Ctrl Pts',(16.6170202186042,19.2003491960952,-3.68841768884857));
#98946=CARTESIAN_POINT('Ctrl Pts',(16.6170599094811,19.1950735078034,-3.6880983937616));
#98947=CARTESIAN_POINT('Ctrl Pts',(16.6176052825337,19.1225828384795,-3.68371111511931));
#98948=CARTESIAN_POINT('Ctrl Pts',(16.6218794874508,19.0499787438806,-3.67932383647702));
#98949=CARTESIAN_POINT('Ctrl Pts',(16.6298970753153,18.9776764428242,-3.67493655783472));
#98950=CARTESIAN_POINT('Ctrl Pts',(16.6379042320844,18.9054682089865,-3.67055498715876));
#98951=CARTESIAN_POINT('Ctrl Pts',(16.6496450608728,18.8335614651472,-3.66617341648279));
#98952=CARTESIAN_POINT('Ctrl Pts',(16.6650821233697,18.7623711781888,-3.66179184580682));
#98953=CARTESIAN_POINT('Ctrl Pts',(16.6805014135,18.6912628511164,-3.65741531954139));
#98954=CARTESIAN_POINT('Ctrl Pts',(16.699608383448,18.620869811639,-3.65303879327595));
#98955=CARTESIAN_POINT('Ctrl Pts',(16.7223140614303,18.5515997538967,-3.64866226701052));
#98956=CARTESIAN_POINT('Ctrl Pts',(16.7296427208095,18.5292416169249,-3.64724966570929));
#98957=CARTESIAN_POINT('Ctrl Pts',(16.7373458914714,18.5070003955267,-3.64583706440805));
#98958=CARTESIAN_POINT('Ctrl Pts',(16.7454194503191,18.4848895418526,-3.64442446310682));
#98959=CARTESIAN_POINT('Origin',(18.734,19.211,0.));
#98960=CARTESIAN_POINT('',(16.747777019274,18.4857290362168,-2.84456321874111));
#98961=CARTESIAN_POINT('',(16.7454194666968,18.4848894969994,-3.06515441818778));
#98962=CARTESIAN_POINT('',(16.7454194503191,18.4848895418526,0.));
#98963=CARTESIAN_POINT('Ctrl Pts',(16.7454194666968,18.4848894969994,-3.06515441818778));
#98964=CARTESIAN_POINT('Ctrl Pts',(16.6929878099064,18.6284827539369,-3.07512667887767));
#98965=CARTESIAN_POINT('Ctrl Pts',(16.6562469357021,18.7773756907385,-3.08537382465129));
#98966=CARTESIAN_POINT('Ctrl Pts',(16.6280919214672,18.9868385248522,-3.09899374936203));
#98967=CARTESIAN_POINT('Ctrl Pts',(16.6227108915773,19.0449985907553,-3.1026987833764));
#98968=CARTESIAN_POINT('Ctrl Pts',(16.6179213236954,19.1390322893946,-3.10855847142046));
#98969=CARTESIAN_POINT('Ctrl Pts',(16.6170073709064,19.1747954552044,-3.11075697795693));
#98970=CARTESIAN_POINT('Ctrl Pts',(16.6169977968628,19.2215398079568,-3.11359306368755));
#98971=CARTESIAN_POINT('Ctrl Pts',(16.6170808697603,19.2325132230707,-3.11425616031307));
#98972=CARTESIAN_POINT('Ctrl Pts',(16.617355670962,19.2504191432636,-3.1153339095973));
#98973=CARTESIAN_POINT('Ctrl Pts',(16.6174961453267,19.2573521244129,-3.11575016009385));
#98974=CARTESIAN_POINT('Ctrl Pts',(16.6178328490843,19.2707252061193,-3.11655110005955));
#98975=CARTESIAN_POINT('Ctrl Pts',(16.6180244187625,19.277165337481,-3.11693593097546));
#98976=CARTESIAN_POINT('Ctrl Pts',(16.6185373490306,19.2921125355497,-3.11782710282682));
#98977=CARTESIAN_POINT('Ctrl Pts',(16.6188806300209,19.3006187761529,-3.11833275166139));
#98978=CARTESIAN_POINT('Ctrl Pts',(16.6201365681075,19.3276865230197,-3.11993714976034));
#98979=CARTESIAN_POINT('Ctrl Pts',(16.6212423395125,19.3462385078596,-3.12102984838258));
#98980=CARTESIAN_POINT('Ctrl Pts',(16.6243860789557,19.3894039111221,-3.1235575311596));
#98981=CARTESIAN_POINT('Ctrl Pts',(16.6266107585169,19.4140012503967,-3.12498671235796));
#98982=CARTESIAN_POINT('Ctrl Pts',(16.6359173822974,19.500081504802,-3.12995531109658));
#98983=CARTESIAN_POINT('Ctrl Pts',(16.6452643348431,19.5612898374677,-3.13342814759911));
#98984=CARTESIAN_POINT('Ctrl Pts',(16.6848813491744,19.761466335755,-3.14471622121767));
#98985=CARTESIAN_POINT('Ctrl Pts',(16.7264585002196,19.8977860910206,-3.15226965910077));
#98986=CARTESIAN_POINT('Ctrl Pts',(16.8104677901499,20.0983446659418,-3.16430892628748));
#98987=CARTESIAN_POINT('Ctrl Pts',(16.843234173352,20.1661747264976,-3.16856359966033));
#98988=CARTESIAN_POINT('Ctrl Pts',(16.8841143625527,20.2404183467846,-3.17358676593651));
#98989=CARTESIAN_POINT('Ctrl Pts',(16.8887460408186,20.2486978475829,-3.17415226598364));
#98990=CARTESIAN_POINT('Ctrl Pts',(16.8956954201968,20.260926777631,-3.17499586404308));
#98991=CARTESIAN_POINT('Ctrl Pts',(16.8979706121172,20.2649003996768,-3.17527129619235));
#98992=CARTESIAN_POINT('Ctrl Pts',(16.9020434239784,20.2719603482061,-3.17576306214405));
#98993=CARTESIAN_POINT('Ctrl Pts',(16.9038359804333,20.2750495374494,-3.1759790676145));
#98994=CARTESIAN_POINT('Ctrl Pts',(16.9077088521027,20.2816850829863,-3.17644483962914));
#98995=CARTESIAN_POINT('Ctrl Pts',(16.9097916527238,20.2852298678033,-3.17669476225511));
#98996=CARTESIAN_POINT('Ctrl Pts',(16.9155744449446,20.2950064697784,-3.17738705526196));
#98997=CARTESIAN_POINT('Ctrl Pts',(16.9192960918719,20.3012253198887,-3.17783080001669));
#98998=CARTESIAN_POINT('Ctrl Pts',(16.9399457208506,20.3353320402637,-3.18028260193025));
#98999=CARTESIAN_POINT('Ctrl Pts',(16.9574836888723,20.362843226496,-3.18232719728519));
#99000=CARTESIAN_POINT('Ctrl Pts',(17.0662162861242,20.5250148758663,-3.1947350877816));
#99001=CARTESIAN_POINT('Ctrl Pts',(17.1720438520995,20.6492039298558,-3.20568688624845));
#99002=CARTESIAN_POINT('Ctrl Pts',(17.3764983259566,20.8396550051589,-3.22393798224768));
#99003=CARTESIAN_POINT('Ctrl Pts',(17.4684036692153,20.9120589788882,-3.23137710151106));
#99004=CARTESIAN_POINT('Ctrl Pts',(17.5777443358775,20.9844052032281,-3.23938255686668));
#99005=CARTESIAN_POINT('Ctrl Pts',(17.5897407225571,20.9921692500584,-3.2402505119227));
#99006=CARTESIAN_POINT('Ctrl Pts',(17.608958800475,21.004332868292,-3.24162479368793));
#99007=CARTESIAN_POINT('Ctrl Pts',(17.6161296672528,21.0088115584032,-3.24213404828691));
#99008=CARTESIAN_POINT('Ctrl Pts',(17.6288239822849,21.0166346969632,-3.24302941946336));
#99009=CARTESIAN_POINT('Ctrl Pts',(17.6343362260356,21.0199970355623,-3.24341619213557));
#99010=CARTESIAN_POINT('Ctrl Pts',(17.6457691799304,21.026899299525,-3.24421426229817));
#99011=CARTESIAN_POINT('Ctrl Pts',(17.6516919886846,21.0304356141779,-3.24462542439077));
#99012=CARTESIAN_POINT('Ctrl Pts',(17.6669394893455,21.0394385955014,-3.24567814733697));
#99013=CARTESIAN_POINT('Ctrl Pts',(17.6762890277062,21.0448629546849,-3.24631816681371));
#99014=CARTESIAN_POINT('Ctrl Pts',(17.7154849602121,21.0672039394384,-3.24897893555428));
#99015=CARTESIAN_POINT('Ctrl Pts',(17.7456997772362,21.083465972287,-3.25097615374836));
#99016=CARTESIAN_POINT('Ctrl Pts',(17.8254447987032,21.1239175083262,-3.25612051576821));
#99017=CARTESIAN_POINT('Ctrl Pts',(17.8755487132813,21.1469204480803,-3.25922826489179));
#99018=CARTESIAN_POINT('Ctrl Pts',(18.0275780243382,21.209653112275,-3.26837300717717));
#99019=CARTESIAN_POINT('Ctrl Pts',(18.1317424662785,21.2434696842161,-3.27426127206076));
#99020=CARTESIAN_POINT('Ctrl Pts',(18.2827868088843,21.2798675645777,-3.28272016865566));
#99021=CARTESIAN_POINT('Ctrl Pts',(18.3278592402491,21.2891856953231,-3.28523622204361));
#99022=CARTESIAN_POINT('Ctrl Pts',(18.3949987144338,21.300798223752,-3.28901509046505));
#99023=CARTESIAN_POINT('Ctrl Pts',(18.4168566471958,21.3042268233531,-3.29025018981404));
#99024=CARTESIAN_POINT('Ctrl Pts',(18.4897453002247,21.3144921709329,-3.29439629947441));
#99025=CARTESIAN_POINT('Ctrl Pts',(18.5409674567388,21.3198094231568,-3.29735448844211));
#99026=CARTESIAN_POINT('Ctrl Pts',(18.6009478783508,21.3238324055423,-3.30092248011162));
#99027=CARTESIAN_POINT('Ctrl Pts',(18.6095713038437,21.3243577867427,-3.30143795753021));
#99028=CARTESIAN_POINT('Ctrl Pts',(18.622656661426,21.3250746449514,-3.30222427639916));
#99029=CARTESIAN_POINT('Ctrl Pts',(18.6271165012822,21.3253048172704,-3.30249300097944));
#99030=CARTESIAN_POINT('Ctrl Pts',(18.6351357008699,21.3256932506871,-3.30297755066702));
#99031=CARTESIAN_POINT('Ctrl Pts',(18.6386947577369,21.3258566392622,-3.30319308557753));
#99032=CARTESIAN_POINT('Ctrl Pts',(18.646443745119,21.3261927777671,-3.30366342433517));
#99033=CARTESIAN_POINT('Ctrl Pts',(18.6506337280332,21.3263620609441,-3.30391841435706));
#99034=CARTESIAN_POINT('Ctrl Pts',(18.6624420011046,21.3268039998604,-3.30463887000105));
#99035=CARTESIAN_POINT('Ctrl Pts',(18.6700612102549,21.3270479531758,-3.30510589555819));
#99036=CARTESIAN_POINT('Ctrl Pts',(18.7164059381543,21.3282812987535,-3.30795906396363));
#99037=CARTESIAN_POINT('Ctrl Pts',(18.7551486955895,21.3282486730973,-3.31039691276878));
#99038=CARTESIAN_POINT('Ctrl Pts',(18.8845059450356,21.3245891696571,-3.31866548505668));
#99039=CARTESIAN_POINT('Ctrl Pts',(18.97488229698,21.3162042498079,-3.3246500656955));
#99040=CARTESIAN_POINT('Ctrl Pts',(19.130734388154,21.2915758828464,-3.33507696129625));
#99041=CARTESIAN_POINT('Ctrl Pts',(19.196498625389,21.2779518004067,-3.33951152027783));
#99042=CARTESIAN_POINT('Ctrl Pts',(19.3726434450192,21.2326312034525,-3.35138282706485));
#99043=CARTESIAN_POINT('Ctrl Pts',(19.4812852787277,21.1950439273391,-3.35868683075174));
#99044=CARTESIAN_POINT('Ctrl Pts',(19.5994118731489,21.1430855619597,-3.36656623016451));
#99045=CARTESIAN_POINT('Ctrl Pts',(19.6124062756236,21.1372125426555,-3.36743235935875));
#99046=CARTESIAN_POINT('Ctrl Pts',(19.6330013126163,21.1276525432891,-3.36880430551127));
#99047=CARTESIAN_POINT('Ctrl Pts',(19.6406407598762,21.1240506704065,-3.36931303489598));
#99048=CARTESIAN_POINT('Ctrl Pts',(19.6540808124361,21.1176153176316,-3.37020779533655));
#99049=CARTESIAN_POINT('Ctrl Pts',(19.659890357605,21.1148008609008,-3.37059447967014));
#99050=CARTESIAN_POINT('Ctrl Pts',(19.6718842843063,21.1089224698088,-3.37139266734787));
#99051=CARTESIAN_POINT('Ctrl Pts',(19.6780667449575,21.1058547741063,-3.37180403381585));
#99052=CARTESIAN_POINT('Ctrl Pts',(19.6939072246733,21.0978980620105,-3.37285790143912));
#99053=CARTESIAN_POINT('Ctrl Pts',(19.7035430228559,21.0929650660462,-3.37349885463178));
#99054=CARTESIAN_POINT('Ctrl Pts',(19.743680942859,21.0720265769892,-3.3761687142773));
#99055=CARTESIAN_POINT('Ctrl Pts',(19.773828973,21.0553512226515,-3.37817388393533));
#99056=CARTESIAN_POINT('Ctrl Pts',(19.8513820324026,21.0099489752026,-3.38334337695911));
#99057=CARTESIAN_POINT('Ctrl Pts',(19.898090490426,20.9800828150596,-3.38646779892359));
#99058=CARTESIAN_POINT('Ctrl Pts',(20.0335281682329,20.8857921549217,-3.39564161633733));
#99059=CARTESIAN_POINT('Ctrl Pts',(20.1184836985275,20.8162750431441,-3.4015423837091));
#99060=CARTESIAN_POINT('Ctrl Pts',(20.2426868186299,20.6974167549793,-3.4109034341488));
#99061=CARTESIAN_POINT('Ctrl Pts',(20.2857741169622,20.6523767865316,-3.41431572028435));
#99062=CARTESIAN_POINT('Ctrl Pts',(20.3638815131606,20.563162131561,-3.42096827558358));
#99063=CARTESIAN_POINT('Ctrl Pts',(20.3992460553724,20.5193617903362,-3.4241908487252));
#99064=CARTESIAN_POINT('Ctrl Pts',(20.4380912279551,20.4671210567527,-3.42805321900816));
#99065=CARTESIAN_POINT('Ctrl Pts',(20.4433173594533,20.4600000724333,-3.42858009519152));
#99066=CARTESIAN_POINT('Ctrl Pts',(20.451142771871,20.4491962760847,-3.4293803964736));
#99067=CARTESIAN_POINT('Ctrl Pts',(20.4537751790517,20.4455374233911,-3.42965159017405));
#99068=CARTESIAN_POINT('Ctrl Pts',(20.4584690077531,20.4389691996341,-3.43013876793881));
#99069=CARTESIAN_POINT('Ctrl Pts',(20.4605347811103,20.4360630038037,-3.43035444773612));
#99070=CARTESIAN_POINT('Ctrl Pts',(20.4649957423871,20.4297534856831,-3.43082297701288));
#99071=CARTESIAN_POINT('Ctrl Pts',(20.4673882075464,20.4263483616963,-3.43107600108407));
#99072=CARTESIAN_POINT('Ctrl Pts',(20.4740508688877,20.4168059029012,-3.43178548864634));
#99073=CARTESIAN_POINT('Ctrl Pts',(20.4782985653936,20.4106530384743,-3.43224343855026));
#99074=CARTESIAN_POINT('Ctrl Pts',(20.5029238557443,20.3745755774155,-3.43493081986129));
#99075=CARTESIAN_POINT('Ctrl Pts',(20.5225624087132,20.3441565994983,-3.43720536256098));
#99076=CARTESIAN_POINT('Ctrl Pts',(20.5834735755453,20.2442778772683,-3.44466394771567));
#99077=CARTESIAN_POINT('Ctrl Pts',(20.621551733202,20.1729575852527,-3.44997280347107));
#99078=CARTESIAN_POINT('Ctrl Pts',(20.732935031487,19.9321198290709,-3.46749316358894));
#99079=CARTESIAN_POINT('Ctrl Pts',(20.7881876152504,19.7551465797868,-3.47965034010632));
#99080=CARTESIAN_POINT('Ctrl Pts',(20.8235802099429,19.5513478117612,-3.49237241659951));
#99081=CARTESIAN_POINT('Ctrl Pts',(20.8270353053704,19.5294106722129,-3.4937272997619));
#99082=CARTESIAN_POINT('Ctrl Pts',(20.8313312895463,19.4990317271568,-3.49558415685693));
#99083=CARTESIAN_POINT('Ctrl Pts',(20.8324674835906,19.4906337560797,-3.49609542916909));
#99084=CARTESIAN_POINT('Ctrl Pts',(20.8343324616095,19.4761971755608,-3.4969708976316));
#99085=CARTESIAN_POINT('Ctrl Pts',(20.8350856984129,19.4701618805719,-3.49733586248594));
#99086=CARTESIAN_POINT('Ctrl Pts',(20.8365837569957,19.4577227334541,-3.49808599021959));
#99087=CARTESIAN_POINT('Ctrl Pts',(20.837325357055,19.4513185514561,-3.49847104774548));
#99088=CARTESIAN_POINT('Ctrl Pts',(20.8389812154041,19.4364240488768,-3.49936399356953));
#99089=CARTESIAN_POINT('Ctrl Pts',(20.839873384816,19.4279313472028,-3.49987118096662));
#99090=CARTESIAN_POINT('Ctrl Pts',(20.8425578397165,19.4007985576625,-3.5014854649064));
#99091=CARTESIAN_POINT('Ctrl Pts',(20.8441542370115,19.3821396660465,-3.50258640332619));
#99092=CARTESIAN_POINT('Ctrl Pts',(20.8472985949722,19.3385921680564,-3.50513595017191));
#99093=CARTESIAN_POINT('Ctrl Pts',(20.8486548380721,19.3136922688832,-3.50657861369475));
#99094=CARTESIAN_POINT('Ctrl Pts',(20.8518764894577,19.2260578491885,-3.51160944547749));
#99095=CARTESIAN_POINT('Ctrl Pts',(20.8513922858796,19.1632677994925,-3.51512908724445));
#99096=CARTESIAN_POINT('Ctrl Pts',(20.8429335710268,19.0013039643041,-3.52409522285026));
#99097=CARTESIAN_POINT('Ctrl Pts',(20.8307606992863,18.9025064183191,-3.52945117451298));
#99098=CARTESIAN_POINT('Ctrl Pts',(20.7979299445984,18.7345249330378,-3.53877346953323));
#99099=CARTESIAN_POINT('Ctrl Pts',(20.7806006530245,18.6648683175245,-3.54270751075005));
#99100=CARTESIAN_POINT('Ctrl Pts',(20.746278597417,18.5517712854519,-3.54939451847304));
#99101=CARTESIAN_POINT('Ctrl Pts',(20.7313275221603,18.5077719279041,-3.55207382890925));
#99102=CARTESIAN_POINT('Ctrl Pts',(20.7122407784917,18.4571358877466,-3.55528720006793));
#99103=CARTESIAN_POINT('Ctrl Pts',(20.7095001066211,18.4499829159889,-3.55574420043702));
#99104=CARTESIAN_POINT('Ctrl Pts',(20.7050447920928,18.4385410944547,-3.5564803867906));
#99105=CARTESIAN_POINT('Ctrl Pts',(20.7033547993185,18.4342426333353,-3.55675813300646));
#99106=CARTESIAN_POINT('Ctrl Pts',(20.7003282714571,18.4266180917129,-3.55725294406247));
#99107=CARTESIAN_POINT('Ctrl Pts',(20.6989973403463,18.4232898366547,-3.55746966987588));
#99108=CARTESIAN_POINT('Ctrl Pts',(20.6961487975362,18.4162186410653,-3.55793170199208));
#99109=CARTESIAN_POINT('Ctrl Pts',(20.6946289495333,18.4124767168053,-3.55817713696921));
#99110=CARTESIAN_POINT('Ctrl Pts',(20.6904764310727,18.402336382944,-3.55884474831909));
#99111=CARTESIAN_POINT('Ctrl Pts',(20.6878231127795,18.3959465589251,-3.55926814500395));
#99112=CARTESIAN_POINT('Ctrl Pts',(20.6742067489765,18.3636036798431,-3.56142455906846));
#99113=CARTESIAN_POINT('Ctrl Pts',(20.662758277842,18.3378596455277,-3.56318468375243));
#99114=CARTESIAN_POINT('Ctrl Pts',(20.6277132086572,18.2631090341327,-3.56840839404944));
#99115=CARTESIAN_POINT('Ctrl Pts',(20.6027386053463,18.2147760204601,-3.5719306550947));
#99116=CARTESIAN_POINT('Ctrl Pts',(20.5063073786562,18.0445667949262,-3.58473693324005));
#99117=CARTESIAN_POINT('Ctrl Pts',(20.4245498040554,17.9289366811572,-3.59417851851971));
#99118=CARTESIAN_POINT('Ctrl Pts',(20.2729908615203,17.7545465879801,-3.60909205489516));
#99119=CARTESIAN_POINT('Ctrl Pts',(20.2098412776637,17.6905903173306,-3.61474964247142));
#99120=CARTESIAN_POINT('Ctrl Pts',(20.1325788705896,17.6217064082067,-3.62106521154277));
#99121=CARTESIAN_POINT('Ctrl Pts',(20.1222565019068,17.6126818599007,-3.62189756626861));
#99122=CARTESIAN_POINT('Ctrl Pts',(20.1055565795846,17.598365447915,-3.62322622708388));
#99123=CARTESIAN_POINT('Ctrl Pts',(20.0992344913194,17.5930097539416,-3.62372516625509));
#99124=CARTESIAN_POINT('Ctrl Pts',(20.0879503834773,17.5835637626124,-3.62460860917325));
#99125=CARTESIAN_POINT('Ctrl Pts',(20.0830008931566,17.5794587227538,-3.62499371394123));
#99126=CARTESIAN_POINT('Ctrl Pts',(20.0726463945855,17.5709501735711,-3.62579443106882));
#99127=CARTESIAN_POINT('Ctrl Pts',(20.0672381763467,17.5665506788518,-3.62620987780965));
#99128=CARTESIAN_POINT('Ctrl Pts',(20.0531300913197,17.555189336429,-3.62728652046865));
#99129=CARTESIAN_POINT('Ctrl Pts',(20.0443967476758,17.5482692574326,-3.62794603533587));
#99130=CARTESIAN_POINT('Ctrl Pts',(20.0061697385541,17.5184674079985,-3.63080325429072));
#99131=CARTESIAN_POINT('Ctrl Pts',(19.9761273438626,17.4962981800244,-3.63297276085202));
#99132=CARTESIAN_POINT('Ctrl Pts',(19.8946914692653,17.4394681885347,-3.63867130106736));
#99133=CARTESIAN_POINT('Ctrl Pts',(19.8423347859398,17.406249459587,-3.64214884170592));
#99134=CARTESIAN_POINT('Ctrl Pts',(19.7069292251707,17.3284570827204,-3.65078677320553));
#99135=CARTESIAN_POINT('Ctrl Pts',(19.6222240937723,17.2870411500413,-3.65586984781523));
#99136=CARTESIAN_POINT('Ctrl Pts',(19.4210144012457,17.2047908058381,-3.6676944257322));
#99137=CARTESIAN_POINT('Ctrl Pts',(19.3031514036269,17.1682269242903,-3.67444122090718));
#99138=CARTESIAN_POINT('Ctrl Pts',(19.1735739266523,17.1401178492513,-3.68230024978787));
#99139=CARTESIAN_POINT('Ctrl Pts',(19.164335112392,17.1381782993091,-3.68286299825159));
#99140=CARTESIAN_POINT('Ctrl Pts',(19.1506054170072,17.135391701481,-3.68370326877679));
#99141=CARTESIAN_POINT('Ctrl Pts',(19.1461241212043,17.1344972694013,-3.68397815543183));
#99142=CARTESIAN_POINT('Ctrl Pts',(19.1381360136509,17.1329297814439,-3.68446932583529));
#99143=CARTESIAN_POINT('Ctrl Pts',(19.1346303611728,17.1322510819609,-3.68468528434452));
#99144=CARTESIAN_POINT('Ctrl Pts',(19.1270784631141,17.1308088365709,-3.68515138830297));
#99145=CARTESIAN_POINT('Ctrl Pts',(19.1230317608604,17.1300482362757,-3.68540169212611));
#99146=CARTESIAN_POINT('Ctrl Pts',(19.111828676928,17.1279763744941,-3.68609609186472));
#99147=CARTESIAN_POINT('Ctrl Pts',(19.1046677943431,17.1266902062738,-3.68654157567169));
#99148=CARTESIAN_POINT('Ctrl Pts',(19.066176442187,17.1199813922492,-3.68894438159497));
#99149=CARTESIAN_POINT('Ctrl Pts',(19.0347352137866,17.1152285224869,-3.6909362948906));
#99150=CARTESIAN_POINT('Ctrl Pts',(18.841308648286,17.0904307994393,-3.70332086242888));
#99151=CARTESIAN_POINT('Ctrl Pts',(18.6775640440237,17.0884676178542,-3.71431350075406));
#99152=CARTESIAN_POINT('Ctrl Pts',(18.3988741370583,17.117423535812,-3.73261642477663));
#99153=CARTESIAN_POINT('Ctrl Pts',(18.2837148017831,17.1391354212299,-3.74006804206649));
#99154=CARTESIAN_POINT('Ctrl Pts',(18.1571460386678,17.1740579896664,-3.7480851297345));
#99155=CARTESIAN_POINT('Ctrl Pts',(18.1434079507728,17.1779986981607,-3.74895323667806));
#99156=CARTESIAN_POINT('Ctrl Pts',(18.1216071999855,17.1844917844461,-3.75032771271529));
#99157=CARTESIAN_POINT('Ctrl Pts',(18.1135182896523,17.1869538198002,-3.75083701098681));
#99158=CARTESIAN_POINT('Ctrl Pts',(18.0992785984693,17.1913813644741,-3.75173243296299));
#99159=CARTESIAN_POINT('Ctrl Pts',(18.0931216938649,17.193326664526,-3.75211921299655));
#99160=CARTESIAN_POINT('Ctrl Pts',(18.0804059895686,17.1974083211125,-3.75291727346725));
#99161=CARTESIAN_POINT('Ctrl Pts',(18.0738485311375,17.1995486285652,-3.75332841862934));
#99162=CARTESIAN_POINT('Ctrl Pts',(18.0570440056722,17.2051245342603,-3.7543810467283));
#99163=CARTESIAN_POINT('Ctrl Pts',(18.0468124943179,17.208606646809,-3.7550209888335));
#99164=CARTESIAN_POINT('Ctrl Pts',(18.0048404161899,17.223250688442,-3.75764269247529));
#99165=CARTESIAN_POINT('Ctrl Pts',(17.9733404272866,17.2350905323301,-3.75960192765196));
#99166=CARTESIAN_POINT('Ctrl Pts',(17.8921203737892,17.2678489390955,-3.76464272767542));
#99167=CARTESIAN_POINT('Ctrl Pts',(17.8428928722314,17.2899258087789,-3.76768663705855));
#99168=CARTESIAN_POINT('Ctrl Pts',(17.6804852539002,17.3703480737555,-3.77777329623982));
#99169=CARTESIAN_POINT('Ctrl Pts',(17.5717401856394,17.4370086425783,-3.78458694596819));
#99170=CARTESIAN_POINT('Ctrl Pts',(17.3877476745824,17.5740153256638,-3.79713120499452));
#99171=CARTESIAN_POINT('Ctrl Pts',(17.3103836803492,17.6408327664611,-3.80279980053515));
#99172=CARTESIAN_POINT('Ctrl Pts',(17.2312943924323,17.7198062591517,-3.80942140215416));
#99173=CARTESIAN_POINT('Ctrl Pts',(17.2244840392838,17.726700679768,-3.80999890105219));
#99174=CARTESIAN_POINT('Ctrl Pts',(17.2144981910691,17.7369495987166,-3.81085699491019));
#99175=CARTESIAN_POINT('Ctrl Pts',(17.2112858430292,17.7402682338026,-3.8111347892569));
#99176=CARTESIAN_POINT('Ctrl Pts',(17.2056059512423,17.7461746121291,-3.81162915001794));
#99177=CARTESIAN_POINT('Ctrl Pts',(17.2031340762655,17.7487581224133,-3.81184537471628));
#99178=CARTESIAN_POINT('Ctrl Pts',(17.1978517144034,17.7543071232828,-3.81230978154288));
#99179=CARTESIAN_POINT('Ctrl Pts',(17.1950433058677,17.7572744463438,-3.8125581101102));
#99180=CARTESIAN_POINT('Ctrl Pts',(17.1892976395439,17.7633805413353,-3.81306905410891));
#99181=CARTESIAN_POINT('Ctrl Pts',(17.1863613188675,17.7665201657942,-3.81333173768555));
#99182=CARTESIAN_POINT('Ctrl Pts',(17.1729076003644,17.7809935002625,-3.81454243739383));
#99183=CARTESIAN_POINT('Ctrl Pts',(17.1625053222708,17.7924329358648,-3.81549866485058));
#99184=CARTESIAN_POINT('Ctrl Pts',(17.0941973456397,17.8692249567763,-3.82190710789897));
#99185=CARTESIAN_POINT('Ctrl Pts',(17.0402625674082,17.9379864944498,-3.82759171384278));
#99186=CARTESIAN_POINT('Ctrl Pts',(16.9494514006864,18.0697861592552,-3.83812735841573));
#99187=CARTESIAN_POINT('Ctrl Pts',(16.9112865256595,18.1317880314201,-3.84295320018642));
#99188=CARTESIAN_POINT('Ctrl Pts',(16.8741060039446,18.1998096180957,-3.84805125711873));
#99189=CARTESIAN_POINT('Ctrl Pts',(16.8718367035901,18.2039947752084,-3.84836416845396));
#99190=CARTESIAN_POINT('Ctrl Pts',(16.8216173512443,18.2973620733673,-3.85532787399593));
#99191=CARTESIAN_POINT('Ctrl Pts',(16.7801280274345,18.3898340573838,-3.86186882407568));
#99192=CARTESIAN_POINT('Ctrl Pts',(16.7454195180457,18.4848893563717,-3.86819359339412));
#99193=CARTESIAN_POINT('',(16.6170008393112,19.2128851108722,-2.8890562790225));
#99194=CARTESIAN_POINT('Ctrl Pts',(16.7454194503191,18.4848895418526,-3.64442446310682));
#99195=CARTESIAN_POINT('Ctrl Pts',(16.7704138790241,18.4164379251386,-3.6400512785945));
#99196=CARTESIAN_POINT('Ctrl Pts',(16.7989618302365,18.3492371530331,-3.63567809408218));
#99197=CARTESIAN_POINT('Ctrl Pts',(16.8309082930386,18.2836753778236,-3.63130490956986));
#99198=CARTESIAN_POINT('Ctrl Pts',(16.8628484348593,18.2181265747783,-3.62693259034326));
#99199=CARTESIAN_POINT('Ctrl Pts',(16.8981855413773,18.1542165580066,-3.62256027111665));
#99200=CARTESIAN_POINT('Ctrl Pts',(16.9367174473244,18.0923112918029,-3.61818795189004));
#99201=CARTESIAN_POINT('Ctrl Pts',(16.9752544398296,18.0303978535473,-3.61381505547797));
#99202=CARTESIAN_POINT('Ctrl Pts',(17.0169868120812,17.9704900994532,-3.60944215906591));
#99203=CARTESIAN_POINT('Ctrl Pts',(17.0616685471728,17.9129258449978,-3.60506926265384));
#99204=CARTESIAN_POINT('Ctrl Pts',(17.1063995662725,17.8552980970997,-3.60069154293171));
#99205=CARTESIAN_POINT('Ctrl Pts',(17.1540861428344,17.80001938801,-3.59631382320958));
#99206=CARTESIAN_POINT('Ctrl Pts',(17.2044419181706,17.7473944949849,-3.59193610348746));
#99207=CARTESIAN_POINT('Ctrl Pts',(17.2548300009133,17.6947358387262,-3.58755557509504));
#99208=CARTESIAN_POINT('Ctrl Pts',(17.3078903391089,17.6447347170448,-3.58317504670262));
#99209=CARTESIAN_POINT('Ctrl Pts',(17.3633016198,17.597657212333,-3.57879451831021));
#99210=CARTESIAN_POINT('Ctrl Pts',(17.418805685217,17.5505008775831,-3.5744066548387));
#99211=CARTESIAN_POINT('Ctrl Pts',(17.4766681650794,17.5062782200529,-3.5700187913672));
#99212=CARTESIAN_POINT('Ctrl Pts',(17.5365374615874,17.4652129370687,-3.56563092789569));
#99213=CARTESIAN_POINT('Ctrl Pts',(17.5579514560577,17.4505247447224,-3.56406148095718));
#99214=CARTESIAN_POINT('Ctrl Pts',(17.5796219550475,17.4362400645932,-3.56249203401867));
#99215=CARTESIAN_POINT('Ctrl Pts',(17.6015321394765,17.4223676887405,-3.56092258708016));
#99216=CARTESIAN_POINT('Ctrl Pts',(17.6627935078071,17.3835802139256,-3.55653437814988));
#99217=CARTESIAN_POINT('Ctrl Pts',(17.7261694924201,17.3478680068777,-3.5521461692196));
#99218=CARTESIAN_POINT('Ctrl Pts',(17.7913186157339,17.3154681992227,-3.54775796028932));
#99219=CARTESIAN_POINT('Ctrl Pts',(17.8563710469468,17.2831164782542,-3.54337626418867));
#99220=CARTESIAN_POINT('Ctrl Pts',(17.9231909643682,17.2540676104731,-3.53899456808802));
#99221=CARTESIAN_POINT('Ctrl Pts',(17.9914091442163,17.22851473627,-3.53461287198737));
#99222=CARTESIAN_POINT('Ctrl Pts',(18.0595471622739,17.2029918887279,-3.53023632472837));
#99223=CARTESIAN_POINT('Ctrl Pts',(18.1290797293046,17.1809570424211,-3.52585977746936));
#99224=CARTESIAN_POINT('Ctrl Pts',(18.199615869865,17.1625560536202,-3.52148323021035));
#99225=CARTESIAN_POINT('Ctrl Pts',(18.2701072774302,17.1441667344591,-3.51710945849401));
#99226=CARTESIAN_POINT('Ctrl Pts',(18.3416005301142,17.1294068217631,-3.51273568677767));
#99227=CARTESIAN_POINT('Ctrl Pts',(18.4136889989947,17.1183724978786,-3.50836191506134));
#99228=CARTESIAN_POINT('Ctrl Pts',(18.485755531112,17.1073415317759,-3.50398947429842));
#99229=CARTESIAN_POINT('Ctrl Pts',(18.5584164432967,17.1000339766644,-3.49961703353551));
#99230=CARTESIAN_POINT('Ctrl Pts',(18.6312560654053,17.0964946952292,-3.4952445927726));
#99231=CARTESIAN_POINT('Ctrl Pts',(18.704097550031,17.0929553232941,-3.4908720402059));
#99232=CARTESIAN_POINT('Ctrl Pts',(18.7771172717469,17.0931844377533,-3.4864994876392));
#99233=CARTESIAN_POINT('Ctrl Pts',(18.8498972932262,17.0971748375462,-3.4821269350725));
#99234=CARTESIAN_POINT('Ctrl Pts',(18.9227528485569,17.1011693787265,-3.47774984450582));
#99235=CARTESIAN_POINT('Ctrl Pts',(18.9953677242803,17.1089329725837,-3.47337275393914));
#99236=CARTESIAN_POINT('Ctrl Pts',(19.0673276840485,17.120406386921,-3.46899566337246));
#99237=CARTESIAN_POINT('Ctrl Pts',(19.1393269438215,17.1318860673157,-3.46461618231416));
#99238=CARTESIAN_POINT('Ctrl Pts',(19.2106701033895,17.1470795015322,-3.46023670125586));
#99239=CARTESIAN_POINT('Ctrl Pts',(19.2809543980013,17.1658765595918,-3.45585722019757));
#99240=CARTESIAN_POINT('Ctrl Pts',(19.3513632710535,17.1847069353106,-3.45146997653849));
#99241=CARTESIAN_POINT('Ctrl Pts',(19.4207090718562,17.2071535415653,-3.44708273287941));
#99242=CARTESIAN_POINT('Ctrl Pts',(19.4886059995035,17.2330569306693,-3.44269548922033));
#99243=CARTESIAN_POINT('Ctrl Pts',(19.5347693678666,17.2506687392518,-3.43971258627979));
#99244=CARTESIAN_POINT('Ctrl Pts',(19.5802633709747,17.2698774944523,-3.43672968333926));
#99245=CARTESIAN_POINT('Ctrl Pts',(19.6249733426257,17.2906210002371,-3.43374678039872));
#99246=CARTESIAN_POINT('Ctrl Pts',(19.690747087516,17.3211371917541,-3.4293585714646));
#99247=CARTESIAN_POINT('Ctrl Pts',(19.7550796205686,17.3550960250398,-3.42497036253047));
#99248=CARTESIAN_POINT('Ctrl Pts',(19.8175867162744,17.3923387263392,-3.42058215359634));
#99249=CARTESIAN_POINT('Ctrl Pts',(19.8800010410865,17.429526153295,-3.41620045749183));
#99250=CARTESIAN_POINT('Ctrl Pts',(19.9405948958129,17.4699875282328,-3.41181876138732));
#99251=CARTESIAN_POINT('Ctrl Pts',(19.9990060261197,17.513516935613,-3.40743706528282));
#99252=CARTESIAN_POINT('Ctrl Pts',(20.0573485186999,17.5569951924752,-3.40306051801994));
#99253=CARTESIAN_POINT('Ctrl Pts',(20.1135129971337,17.6035340332493,-3.39868397075707));
#99254=CARTESIAN_POINT('Ctrl Pts',(20.1671651917876,17.6528836586929,-3.39430742349419));
#99255=CARTESIAN_POINT('Ctrl Pts',(20.2207833609995,17.7022019873212,-3.38993365177399));
#99256=CARTESIAN_POINT('Ctrl Pts',(20.2718920534962,17.7543272380349,-3.38555988005378));
#99257=CARTESIAN_POINT('Ctrl Pts',(20.3201902946222,17.8089695619402,-3.38118610833357));
#99258=CARTESIAN_POINT('Ctrl Pts',(20.3684738384312,17.8635952580027,-3.3768136675668));
#99259=CARTESIAN_POINT('Ctrl Pts',(20.413948309491,17.9207361453916,-3.37244122680002));
#99260=CARTESIAN_POINT('Ctrl Pts',(20.4563509910177,17.9800669946174,-3.36806878603325));
#99261=CARTESIAN_POINT('Ctrl Pts',(20.4987547567856,18.0393993609393,-3.36369623346269));
#99262=CARTESIAN_POINT('Ctrl Pts',(20.5380862982224,18.10092140666,-3.35932368089214));
#99263=CARTESIAN_POINT('Ctrl Pts',(20.5741254487323,18.1642778148296,-3.35495112832159));
#99264=CARTESIAN_POINT('Ctrl Pts',(20.6102020020315,18.2276999766687,-3.35057403775109));
#99265=CARTESIAN_POINT('Ctrl Pts',(20.6429791031824,18.2929598817764,-3.34619694718059));
#99266=CARTESIAN_POINT('Ctrl Pts',(20.6722823388101,18.3596771616732,-3.3418198566101));
#99267=CARTESIAN_POINT('Ctrl Pts',(20.7016015780223,18.4264308783525,-3.33744037554801));
#99268=CARTESIAN_POINT('Ctrl Pts',(20.7274430033813,18.4946431030975,-3.33306089448592));
#99269=CARTESIAN_POINT('Ctrl Pts',(20.7496812078501,18.5639155632221,-3.32868141342383));
#99270=CARTESIAN_POINT('Ctrl Pts',(20.7719588293866,18.6333108083162,-3.32429416976102));
#99271=CARTESIAN_POINT('Ctrl Pts',(20.7906203524711,18.7037695748855,-3.31990692609822));
#99272=CARTESIAN_POINT('Ctrl Pts',(20.8055910206616,18.7748811594138,-3.31551968243541));
#99273=CARTESIAN_POINT('Ctrl Pts',(20.8157696323556,18.8232301840966,-3.31253677952937));
#99274=CARTESIAN_POINT('Ctrl Pts',(20.8242431499885,18.8718807754378,-3.30955387662333));
#99275=CARTESIAN_POINT('Ctrl Pts',(20.8310018039417,18.9207028517787,-3.30657097371729));
#99276=CARTESIAN_POINT('Ctrl Pts',(20.8409445967654,18.9925259978733,-3.30218276479086));
#99277=CARTESIAN_POINT('Ctrl Pts',(20.8472125720511,19.0650007495843,-3.29779455586443));
#99278=CARTESIAN_POINT('Ctrl Pts',(20.8497312594192,19.1377180928425,-3.29340634693799));
#99279=CARTESIAN_POINT('Ctrl Pts',(20.8522462086376,19.2103275115067,-3.28902465084118));
#99280=CARTESIAN_POINT('Ctrl Pts',(20.8510228997994,19.2831783288738,-3.28464295474436));
#99281=CARTESIAN_POINT('Ctrl Pts',(20.8460383938858,19.355854488202,-3.28026125864754));
#99282=CARTESIAN_POINT('Ctrl Pts',(20.8410597451634,19.4284452472597,-3.27588471139231));
#99283=CARTESIAN_POINT('Ctrl Pts',(20.8323287119824,19.5008612771246,-3.27150816413708));
#99284=CARTESIAN_POINT('Ctrl Pts',(20.8198744021611,19.5726862983432,-3.26713161688185));
#99285=CARTESIAN_POINT('Ctrl Pts',(20.8074279906819,19.6444657691777,-3.26275784516926));
#99286=CARTESIAN_POINT('Ctrl Pts',(20.7912630697951,19.7156545009196,-3.25838407345667));
#99287=CARTESIAN_POINT('Ctrl Pts',(20.7714604446778,19.7858425318062,-3.25401030174408));
#99288=CARTESIAN_POINT('Ctrl Pts',(20.7516638455656,19.8560092042398,-3.24963786098487));
#99289=CARTESIAN_POINT('Ctrl Pts',(20.7282318707952,19.9251753164025,-3.24526542022567));
#99290=CARTESIAN_POINT('Ctrl Pts',(20.7012957832859,19.992943924502,-3.24089297946647));
#99291=CARTESIAN_POINT('Ctrl Pts',(20.6743590070176,20.0607142654529,-3.23652042690343));
#99292=CARTESIAN_POINT('Ctrl Pts',(20.6439181201481,20.1270865838657,-3.2321478743404));
#99293=CARTESIAN_POINT('Ctrl Pts',(20.6101527159991,20.1916834281506,-3.22777532177736));
#99294=CARTESIAN_POINT('Ctrl Pts',(20.5763522688394,20.2563473134783,-3.22339823121425));
#99295=CARTESIAN_POINT('Ctrl Pts',(20.5392206395603,20.3192316172821,-3.21902114065115));
#99296=CARTESIAN_POINT('Ctrl Pts',(20.4989832512063,20.3799837992723,-3.21464405008804));
#99297=CARTESIAN_POINT('Ctrl Pts',(20.4587238877208,20.4407691602846,-3.21026456903327));
#99298=CARTESIAN_POINT('Ctrl Pts',(20.4153556750978,20.4994196929838,-3.20588508797851));
#99299=CARTESIAN_POINT('Ctrl Pts',(20.3691456171873,20.5556143724478,-3.20150560692374));
#99300=CARTESIAN_POINT('Ctrl Pts',(20.322853652258,20.6119086566055,-3.19711836326808));
#99301=CARTESIAN_POINT('Ctrl Pts',(20.2737101085746,20.6657380382375,-3.19273111961242));
#99302=CARTESIAN_POINT('Ctrl Pts',(20.2220198585544,20.716817352984,-3.18834387595676));
#99303=CARTESIAN_POINT('Ctrl Pts',(20.1868754689114,20.7515463655046,-3.18536097298313));
#99304=CARTESIAN_POINT('Ctrl Pts',(20.1505545743034,20.7850048960123,-3.1823780700095));
#99305=CARTESIAN_POINT('Ctrl Pts',(20.1131612647175,20.8171143190642,-3.17939516703586));
#99306=CARTESIAN_POINT('Ctrl Pts',(20.0581512102736,20.8643511411,-3.17500695810766));
#99307=CARTESIAN_POINT('Ctrl Pts',(20.000604149589,20.9088507248998,-3.17061874917945));
#99308=CARTESIAN_POINT('Ctrl Pts',(19.9408236893637,20.9503290611011,-3.16623054025124));
#99309=CARTESIAN_POINT('Ctrl Pts',(19.8811319532539,20.9917458365736,-3.16184884415272));
#99310=CARTESIAN_POINT('Ctrl Pts',(19.8192137908515,21.0301499931512,-3.1574671480542));
#99311=CARTESIAN_POINT('Ctrl Pts',(19.7554066235781,21.0652970391258,-3.15308545195568));
#99312=CARTESIAN_POINT('Ctrl Pts',(19.6916744348053,21.1004027845237,-3.14870890469886));
#99313=CARTESIAN_POINT('Ctrl Pts',(19.6260580710932,21.1322587908208,-3.14433235744203));
#99314=CARTESIAN_POINT('Ctrl Pts',(19.5589233130942,21.1606642089123,-3.13995581018521));
#99315=CARTESIAN_POINT('Ctrl Pts',(19.4918311309836,21.1890516127003,-3.1355820384711));
#99316=CARTESIAN_POINT('Ctrl Pts',(19.423222908347,21.2139925826756,-3.13120826675699));
#99317=CARTESIAN_POINT('Ctrl Pts',(19.3534870964587,21.2353331586775,-3.12683449504287));
#99318=CARTESIAN_POINT('Ctrl Pts',(19.2837725054128,21.2566672406702,-3.12246205428222));
#99319=CARTESIAN_POINT('Ctrl Pts',(19.2129314673179,21.2744029627461,-3.11808961352157));
#99320=CARTESIAN_POINT('Ctrl Pts',(19.1413687992146,21.288435838101,-3.11371717276091));
#99321=CARTESIAN_POINT('Ctrl Pts',(19.0698043012465,21.302469072278,-3.1093446201965));
#99322=CARTESIAN_POINT('Ctrl Pts',(18.9975186103822,21.312799180891,-3.10497206763209));
#99323=CARTESIAN_POINT('Ctrl Pts',(18.9249263141349,21.3193728661152,-3.10059951506768));
#99324=CARTESIAN_POINT('Ctrl Pts',(18.8522586788649,21.3259533737578,-3.09622242450331));
#99325=CARTESIAN_POINT('Ctrl Pts',(18.7792842843306,21.3287696306808,-3.09184533393895));
#99326=CARTESIAN_POINT('Ctrl Pts',(18.7064215783433,21.3278203586178,-3.08746824337459));
#99327=CARTESIAN_POINT('Ctrl Pts',(18.6335190793282,21.3268705681222,-3.08308876231863));
#99328=CARTESIAN_POINT('Ctrl Pts',(18.5607288720058,21.3221511854103,-3.07870928126267));
#99329=CARTESIAN_POINT('Ctrl Pts',(18.4884654116523,21.3137129537635,-3.07432980020672));
#99330=CARTESIAN_POINT('Ctrl Pts',(18.4160738648003,21.3052597654078,-3.06994255654998));
#99331=CARTESIAN_POINT('Ctrl Pts',(18.3442114053975,21.2930746456032,-3.06555531289325));
#99332=CARTESIAN_POINT('Ctrl Pts',(18.2732828331998,21.2772595897456,-3.06116806923651));
#99333=CARTESIAN_POINT('Ctrl Pts',(18.225058238315,21.266506875597,-3.05818516627582));
#99334=CARTESIAN_POINT('Ctrl Pts',(18.1772650979176,21.2540772191558,-3.05520226331512));
#99335=CARTESIAN_POINT('Ctrl Pts',(18.1300258654965,21.2400155851671,-3.05221936035442));
#99336=CARTESIAN_POINT('Ctrl Pts',(18.0605312740272,21.2193292306402,-3.04783115140135));
#99337=CARTESIAN_POINT('Ctrl Pts',(17.9919650333991,21.1950280401746,-3.04344294244829));
#99338=CARTESIAN_POINT('Ctrl Pts',(17.9247302870924,21.1672135700813,-3.03905473349522));
#99339=CARTESIAN_POINT('Ctrl Pts',(17.8575953282952,21.1394403812727,-3.03467303737171));
#99340=CARTESIAN_POINT('Ctrl Pts',(17.791788382932,21.1081644467877,-3.0302913412482));
#99341=CARTESIAN_POINT('Ctrl Pts',(17.7276976696562,21.0735371459235,-3.02590964512469));
#99342=CARTESIAN_POINT('Ctrl Pts',(17.6636822680688,21.0389505348933,-3.02153309784281));
#99343=CARTESIAN_POINT('Ctrl Pts',(17.6013795146524,21.0010206087461,-3.01715655056093));
#99344=CARTESIAN_POINT('Ctrl Pts',(17.5411562818512,20.9599462153173,-3.01278000327905));
#99345=CARTESIAN_POINT('Ctrl Pts',(17.4809712417489,20.918897870672,-3.00840623153985));
#99346=CARTESIAN_POINT('Ctrl Pts',(17.4228635031208,20.8747092865794,-3.00403245980065));
#99347=CARTESIAN_POINT('Ctrl Pts',(17.367172783407,20.8276237533764,-2.99965868806145));
#99348=CARTESIAN_POINT('Ctrl Pts',(17.3114990105668,20.7805525484596,-2.99528624727572));
#99349=CARTESIAN_POINT('Ctrl Pts',(17.2582411645738,20.7305864558404,-2.99091380648998));
#99350=CARTESIAN_POINT('Ctrl Pts',(17.2077062220831,20.6780093058642,-2.98654136570425));
#99351=CARTESIAN_POINT('Ctrl Pts',(17.1571699874092,20.6254308114853,-2.9821688131148));
#99352=CARTESIAN_POINT('Ctrl Pts',(17.1093571273009,20.5702414763594,-2.97779626052535));
#99353=CARTESIAN_POINT('Ctrl Pts',(17.064536865154,20.5127610538767,-2.9734237079359));
#99354=CARTESIAN_POINT('Ctrl Pts',(17.0196700868515,20.4552209760473,-2.96904661734673));
#99355=CARTESIAN_POINT('Ctrl Pts',(16.9778024047636,20.3953854446857,-2.96466952675757));
#99356=CARTESIAN_POINT('Ctrl Pts',(16.9391613915757,20.3336056162827,-2.96029243616841));
#99357=CARTESIAN_POINT('Ctrl Pts',(16.9004992750975,20.2717920476242,-2.95591295508774));
#99358=CARTESIAN_POINT('Ctrl Pts',(16.8650675705241,20.2080324897248,-2.95153347400708));
#99359=CARTESIAN_POINT('Ctrl Pts',(16.8330479475686,20.1427029002621,-2.94715399292642));
#99360=CARTESIAN_POINT('Ctrl Pts',(16.8009715700497,20.0772575145475,-2.94276674924541));
#99361=CARTESIAN_POINT('Ctrl Pts',(16.7723195413297,20.0102369839267,-2.93837950556439));
#99362=CARTESIAN_POINT('Ctrl Pts',(16.7472252098539,19.9420368891101,-2.93399226188338));
#99363=CARTESIAN_POINT('Ctrl Pts',(16.7301634837498,19.8956673996836,-2.93100935914658));
#99364=CARTESIAN_POINT('Ctrl Pts',(16.714745338617,19.8487529982297,-2.92802645640979));
#99365=CARTESIAN_POINT('Ctrl Pts',(16.7009992479662,19.8014209872878,-2.92504355367299));
#99366=CARTESIAN_POINT('Ctrl Pts',(16.6758066766592,19.7146752287267,-2.91957676374651));
#99367=CARTESIAN_POINT('Ctrl Pts',(16.6561521069757,19.6262535084973,-2.91410997382002));
#99368=CARTESIAN_POINT('Ctrl Pts',(16.6422180861875,19.5367873923999,-2.90864318389354));
#99369=CARTESIAN_POINT('Ctrl Pts',(16.6285119268963,19.44878430578,-2.90326579177662));
#99370=CARTESIAN_POINT('Ctrl Pts',(16.6203407792486,19.3597706087752,-2.8978883996597));
#99371=CARTESIAN_POINT('Ctrl Pts',(16.6178326248382,19.2703686811429,-2.89251100754278));
#99372=CARTESIAN_POINT('Ctrl Pts',(16.6172955000023,19.2512231311289,-2.89135943136935));
#99373=CARTESIAN_POINT('Ctrl Pts',(16.6170179137274,19.2320598582303,-2.89020785519593));
#99374=CARTESIAN_POINT('Ctrl Pts',(16.6170008393112,19.2128851108722,-2.8890562790225));
#99375=CARTESIAN_POINT('Ctrl Pts',(16.6180380291883,19.2128841872923,-2.8890562790225));
#99376=CARTESIAN_POINT('Ctrl Pts',(16.6201501796595,18.9660536838257,-2.8742252589287));
#99377=CARTESIAN_POINT('Ctrl Pts',(16.6645220593274,18.718557967196,-2.85939423883491));
#99378=CARTESIAN_POINT('Ctrl Pts',(16.747777019274,18.4857290362168,-2.84456321874111));
#99379=CARTESIAN_POINT('Origin',(18.734,19.211,0.));
#99380=CARTESIAN_POINT('',(16.7454194497489,18.4848895434144,-2.04625067101847));
#99381=CARTESIAN_POINT('',(16.7454194503195,18.4848895418517,-2.26547384646959));
#99382=CARTESIAN_POINT('',(16.7454194503191,18.4848895418526,0.));
#99383=CARTESIAN_POINT('',(16.6170007438825,19.2092252893056,-2.31031846004158));
#99384=CARTESIAN_POINT('Ctrl Pts',(16.7454194503191,18.4848895418526,-2.26547384646965));
#99385=CARTESIAN_POINT('Ctrl Pts',(16.7453677674078,18.4850310845493,-2.26548208690514));
#99386=CARTESIAN_POINT('Ctrl Pts',(16.7453160995444,18.4851726329394,-2.26549032756363));
#99387=CARTESIAN_POINT('Ctrl Pts',(16.71039107295,18.5808843594811,-2.27106239636578));
#99388=CARTESIAN_POINT('Ctrl Pts',(16.6824565881579,18.6788318784946,-2.27671183763777));
#99389=CARTESIAN_POINT('Ctrl Pts',(16.6596923791677,18.7878796593165,-2.28331158252327));
#99390=CARTESIAN_POINT('Ctrl Pts',(16.6577771067251,18.7973801045402,-2.28388912020902));
#99391=CARTESIAN_POINT('Ctrl Pts',(16.6550454939141,18.8114271084375,-2.28474726085886));
#99392=CARTESIAN_POINT('Ctrl Pts',(16.6541786621636,18.8159638803859,-2.28502506276829));
#99393=CARTESIAN_POINT('Ctrl Pts',(16.6526671367138,18.824017703857,-2.28551943186517));
#99394=CARTESIAN_POINT('Ctrl Pts',(16.6520164991973,18.8275335901293,-2.28573565729369));
#99395=CARTESIAN_POINT('Ctrl Pts',(16.6506415073593,18.8350703750618,-2.28620005991831));
#99396=CARTESIAN_POINT('Ctrl Pts',(16.6499198953488,18.839091666524,-2.28644838352347));
#99397=CARTESIAN_POINT('Ctrl Pts',(16.6484629280945,18.847348243196,-2.28695931545769));
#99398=CARTESIAN_POINT('Ctrl Pts',(16.647728823752,18.8515837275005,-2.2872219919196));
#99399=CARTESIAN_POINT('Ctrl Pts',(16.6459036982747,18.8623079735055,-2.28788849722442));
#99400=CARTESIAN_POINT('Ctrl Pts',(16.6448300284559,18.8687995878549,-2.28829325045048));
#99401=CARTESIAN_POINT('Ctrl Pts',(16.6260486277417,18.9857393177545,-2.29560661568504));
#99402=CARTESIAN_POINT('Ctrl Pts',(16.6170944893144,19.0973991701253,-2.30293656026631));
#99403=CARTESIAN_POINT('Ctrl Pts',(16.6170007438825,19.2092252893056,-2.31031846004158));
#99404=CARTESIAN_POINT('Ctrl Pts',(16.6170007453236,19.2092235711201,-2.3103183466202));
#99405=CARTESIAN_POINT('Ctrl Pts',(16.616915726726,19.3105416197922,-2.31700658397897));
#99406=CARTESIAN_POINT('Ctrl Pts',(16.6241043877404,19.4117441614251,-2.32371994782463));
#99407=CARTESIAN_POINT('Ctrl Pts',(16.6510544996473,19.5993334501703,-2.33599024637347));
#99408=CARTESIAN_POINT('Ctrl Pts',(16.6690366514094,19.6857574113246,-2.34157366617144));
#99409=CARTESIAN_POINT('Ctrl Pts',(16.6977848563464,19.7906013373736,-2.34824548702124));
#99410=CARTESIAN_POINT('Ctrl Pts',(16.7034969581734,19.8103056525321,-2.34949514501999));
#99411=CARTESIAN_POINT('Ctrl Pts',(16.7120848616136,19.8383967346214,-2.35127113872248));
#99412=CARTESIAN_POINT('Ctrl Pts',(16.7147281849366,19.8468528368021,-2.35180503175381));
#99413=CARTESIAN_POINT('Ctrl Pts',(16.7194026267877,19.8614834108317,-2.3527275766178));
#99414=CARTESIAN_POINT('Ctrl Pts',(16.7214092264388,19.8676655340124,-2.35311702758627));
#99415=CARTESIAN_POINT('Ctrl Pts',(16.7253221591816,19.8795344444876,-2.35386405145122));
#99416=CARTESIAN_POINT('Ctrl Pts',(16.7272242480617,19.8852225554174,-2.35422175979312));
#99417=CARTESIAN_POINT('Ctrl Pts',(16.7322704291892,19.9001023844301,-2.35515676684877));
#99418=CARTESIAN_POINT('Ctrl Pts',(16.7354536847999,19.9092807470241,-2.35573276596104));
#99419=CARTESIAN_POINT('Ctrl Pts',(16.7467207709941,19.9410591482834,-2.35772473922642));
#99420=CARTESIAN_POINT('Ctrl Pts',(16.75512586698,19.9635439049138,-2.3591300440431));
#99421=CARTESIAN_POINT('Ctrl Pts',(16.8192012734972,20.1264516444741,-2.36929205006344));
#99422=CARTESIAN_POINT('Ctrl Pts',(16.8893769880301,20.2607040579724,-2.37751638336487));
#99423=CARTESIAN_POINT('Ctrl Pts',(17.0104437718363,20.4420686199338,-2.38935807424816));
#99424=CARTESIAN_POINT('Ctrl Pts',(17.0502560833175,20.4959832322531,-2.39299171086651));
#99425=CARTESIAN_POINT('Ctrl Pts',(17.1266257048819,20.5897484999617,-2.39967841622019));
#99426=CARTESIAN_POINT('Ctrl Pts',(17.1622799555692,20.6302585571004,-2.40270475103767));
#99427=CARTESIAN_POINT('Ctrl Pts',(17.2186821763871,20.6896078423788,-2.40743001718127));
#99428=CARTESIAN_POINT('Ctrl Pts',(17.2383225651946,20.7094719213274,-2.40906497406223));
#99429=CARTESIAN_POINT('Ctrl Pts',(17.2632324094003,20.7336877807824,-2.41113480030659));
#99430=CARTESIAN_POINT('Ctrl Pts',(17.2681385286067,20.7384113810998,-2.41154228590584));
#99431=CARTESIAN_POINT('Ctrl Pts',(17.276023810327,20.7459303304026,-2.41219709676157));
#99432=CARTESIAN_POINT('Ctrl Pts',(17.2789884673509,20.748740917077,-2.41244326280438));
#99433=CARTESIAN_POINT('Ctrl Pts',(17.2845632807302,20.7539954577843,-2.41290615429137));
#99434=CARTESIAN_POINT('Ctrl Pts',(17.2871715001504,20.7564413859003,-2.41312272352551));
#99435=CARTESIAN_POINT('Ctrl Pts',(17.2931634827415,20.7620320660284,-2.41362025185677));
#99436=CARTESIAN_POINT('Ctrl Pts',(17.2965513410501,20.765172349279,-2.41390154580439));
#99437=CARTESIAN_POINT('Ctrl Pts',(17.307080934092,20.7748685893667,-2.41477571628584));
#99438=CARTESIAN_POINT('Ctrl Pts',(17.3142573268096,20.7813864871993,-2.41537135834745));
#99439=CARTESIAN_POINT('Ctrl Pts',(17.3958893893346,20.8545112186955,-2.42214262180574));
#99440=CARTESIAN_POINT('Ctrl Pts',(17.4749172679588,20.9158093931919,-2.42865320554723));
#99441=CARTESIAN_POINT('Ctrl Pts',(17.6998425835254,21.0660798275081,-2.44647593700132));
#99442=CARTESIAN_POINT('Ctrl Pts',(17.8526864934017,21.14338380602,-2.45780560408483));
#99443=CARTESIAN_POINT('Ctrl Pts',(18.0407436312296,21.2114861330929,-2.47033978586432));
#99444=CARTESIAN_POINT('Ctrl Pts',(18.0685251761512,21.2208986425922,-2.47215989962421));
#99445=CARTESIAN_POINT('Ctrl Pts',(18.1167827612908,21.2361381544597,-2.47526807927265));
#99446=CARTESIAN_POINT('Ctrl Pts',(18.1371670536833,21.242239067777,-2.4765648267941));
#99447=CARTESIAN_POINT('Ctrl Pts',(18.166291081568,21.25047944537,-2.47839524803608));
#99448=CARTESIAN_POINT('Ctrl Pts',(18.1749573133718,21.2528719603782,-2.47893712926988));
#99449=CARTESIAN_POINT('Ctrl Pts',(18.189937141537,21.2569049716091,-2.47986906540596));
#99450=CARTESIAN_POINT('Ctrl Pts',(18.196243511701,21.2585716123213,-2.48025996444069));
#99451=CARTESIAN_POINT('Ctrl Pts',(18.2083351831741,21.2617074697892,-2.48100675098293));
#99452=CARTESIAN_POINT('Ctrl Pts',(18.2141191829561,21.2631814158332,-2.48136278833935));
#99453=CARTESIAN_POINT('Ctrl Pts',(18.2291803387941,21.2669517130647,-2.48228684940491));
#99454=CARTESIAN_POINT('Ctrl Pts',(18.2384670148812,21.2692097565617,-2.48285363310706));
#99455=CARTESIAN_POINT('Ctrl Pts',(18.2702097351164,21.2767006637273,-2.48478101503239));
#99456=CARTESIAN_POINT('Ctrl Pts',(18.2927363233567,21.2816296315469,-2.48613186100627));
#99457=CARTESIAN_POINT('Ctrl Pts',(18.4864623569375,21.3207130051364,-2.49761503257089));
#99458=CARTESIAN_POINT('Ctrl Pts',(18.6611960902983,21.3339390428514,-2.50700554760839));
#99459=CARTESIAN_POINT('Ctrl Pts',(18.9231250715244,21.3213558236439,-2.52127175192693));
#99460=CARTESIAN_POINT('Ctrl Pts',(19.0103131151477,21.3117185972704,-2.5260677647394));
#99461=CARTESIAN_POINT('Ctrl Pts',(19.134067892197,21.2902011619123,-2.53323830618952));
#99462=CARTESIAN_POINT('Ctrl Pts',(19.1713060297255,21.2826888816811,-2.53544442749617));
#99463=CARTESIAN_POINT('Ctrl Pts',(19.2157074006118,21.272481130113,-2.53815504940848));
#99464=CARTESIAN_POINT('Ctrl Pts',(19.223086241022,21.2707429729266,-2.53860819242691));
#99465=CARTESIAN_POINT('Ctrl Pts',(19.2345230353907,21.2679840055428,-2.53931492556288));
#99466=CARTESIAN_POINT('Ctrl Pts',(19.2385876525667,21.2669907120893,-2.53956695956276));
#99467=CARTESIAN_POINT('Ctrl Pts',(19.2461084882052,21.2651291575041,-2.54003494550051));
#99468=CARTESIAN_POINT('Ctrl Pts',(19.2495654691785,21.2642642172432,-2.54025070484568));
#99469=CARTESIAN_POINT('Ctrl Pts',(19.2573611476283,21.2622928015224,-2.54073871236004));
#99470=CARTESIAN_POINT('Ctrl Pts',(19.2616985029387,21.2611812938295,-2.5410112466961));
#99471=CARTESIAN_POINT('Ctrl Pts',(19.2744470798398,21.2578711578748,-2.54181522036926));
#99472=CARTESIAN_POINT('Ctrl Pts',(19.2828482030478,21.2556344971907,-2.54234878117279));
#99473=CARTESIAN_POINT('Ctrl Pts',(19.3421863819696,21.239444627566,-2.54614281721492));
#99474=CARTESIAN_POINT('Ctrl Pts',(19.3925951488972,21.2236424677904,-2.5494984486381));
#99475=CARTESIAN_POINT('Ctrl Pts',(19.4570269869958,21.2007646504455,-2.55391577498353));
#99476=CARTESIAN_POINT('Ctrl Pts',(19.4716402352252,21.1953936742222,-2.55492638070868));
#99477=CARTESIAN_POINT('Ctrl Pts',(19.6180919115667,21.1397253820128,-2.56513472761021));
#99478=CARTESIAN_POINT('Ctrl Pts',(19.7446502528874,21.0765266625902,-2.57458272746252));
#99479=CARTESIAN_POINT('Ctrl Pts',(19.9499321592801,20.9469515977538,-2.59033250513701));
#99480=CARTESIAN_POINT('Ctrl Pts',(20.0318701673413,20.8865766933043,-2.59676211479777));
#99481=CARTESIAN_POINT('Ctrl Pts',(20.1203930948011,20.8109441717258,-2.60386217551483));
#99482=CARTESIAN_POINT('Ctrl Pts',(20.1315224428851,20.8012321229728,-2.60475802605912));
#99483=CARTESIAN_POINT('Ctrl Pts',(20.1483432162397,20.7862404573462,-2.60611719572834));
#99484=CARTESIAN_POINT('Ctrl Pts',(20.1541085918524,20.7810448470131,-2.60658400468454));
#99485=CARTESIAN_POINT('Ctrl Pts',(20.1645471638488,20.7715333300532,-2.60743098057794));
#99486=CARTESIAN_POINT('Ctrl Pts',(20.1692297071773,20.7672278596677,-2.60781158161727));
#99487=CARTESIAN_POINT('Ctrl Pts',(20.1792983518375,20.7578859195777,-2.60863144837453));
#99488=CARTESIAN_POINT('Ctrl Pts',(20.184677700351,20.7528422700866,-2.60907040059836));
#99489=CARTESIAN_POINT('Ctrl Pts',(20.1991959300207,20.7390868093347,-2.61025768541833));
#99490=CARTESIAN_POINT('Ctrl Pts',(20.2082834975006,20.7303210949628,-2.61100368404767));
#99491=CARTESIAN_POINT('Ctrl Pts',(20.2521491909447,20.6872448001146,-2.61461938551674));
#99492=CARTESIAN_POINT('Ctrl Pts',(20.2858125643751,20.6518171230195,-2.61743945916776));
#99493=CARTESIAN_POINT('Ctrl Pts',(20.3452568888793,20.5847544751773,-2.62253173164243));
#99494=CARTESIAN_POINT('Ctrl Pts',(20.3714063039008,20.5534794077522,-2.62481624401318));
#99495=CARTESIAN_POINT('Ctrl Pts',(20.4697864995513,20.4286609130493,-2.63363530300484));
#99496=CARTESIAN_POINT('Ctrl Pts',(20.5350358570186,20.3298936949913,-2.63997299850123));
#99497=CARTESIAN_POINT('Ctrl Pts',(20.6275059368221,20.1606831698113,-2.65050617048442));
#99498=CARTESIAN_POINT('Ctrl Pts',(20.6598146038472,20.0933260463539,-2.65462747392556));
#99499=CARTESIAN_POINT('Ctrl Pts',(20.701757070452,19.992544824345,-2.66088162903481));
#99500=CARTESIAN_POINT('Ctrl Pts',(20.7142361359487,19.9603628877799,-2.66289150203385));
#99501=CARTESIAN_POINT('Ctrl Pts',(20.728418654839,19.9209560378632,-2.66538441873089));
#99502=CARTESIAN_POINT('Ctrl Pts',(20.7308787908355,19.9140067123074,-2.6658252267002));
#99503=CARTESIAN_POINT('Ctrl Pts',(20.7346633078189,19.9031361556126,-2.6665168226936));
#99504=CARTESIAN_POINT('Ctrl Pts',(20.736012598243,19.8992235719312,-2.6667661598703));
#99505=CARTESIAN_POINT('Ctrl Pts',(20.7385037790302,19.8919304895642,-2.66723174114806));
#99506=CARTESIAN_POINT('Ctrl Pts',(20.7396485991476,19.8885510518587,-2.66744780917107));
#99507=CARTESIAN_POINT('Ctrl Pts',(20.7422303640487,19.8808659629102,-2.66793990345803));
#99508=CARTESIAN_POINT('Ctrl Pts',(20.7436620016921,19.8765585935295,-2.66821623705707));
#99509=CARTESIAN_POINT('Ctrl Pts',(20.7478851138569,19.8637146498074,-2.66904170753367));
#99510=CARTESIAN_POINT('Ctrl Pts',(20.7506360864048,19.8551650055277,-2.66959313536422));
#99511=CARTESIAN_POINT('Ctrl Pts',(20.7714940869043,19.7888979320506,-2.67388080436279));
#99512=CARTESIAN_POINT('Ctrl Pts',(20.7871725011374,19.7304510700462,-2.6777416507676));
#99513=CARTESIAN_POINT('Ctrl Pts',(20.8134037128092,19.6127274994457,-2.68557058491372));
#99514=CARTESIAN_POINT('Ctrl Pts',(20.8239744762868,19.5535068930085,-2.68953441005239));
#99515=CARTESIAN_POINT('Ctrl Pts',(20.8465547164529,19.3860612107819,-2.70069675926838));
#99516=CARTESIAN_POINT('Ctrl Pts',(20.8527615264669,19.2772339121808,-2.70788988127502));
#99517=CARTESIAN_POINT('Ctrl Pts',(20.8490659444797,19.0935944048813,-2.71968984222296));
#99518=CARTESIAN_POINT('Ctrl Pts',(20.8435950501378,19.0189091960864,-2.72439711894139));
#99519=CARTESIAN_POINT('Ctrl Pts',(20.8318167920761,18.9260326723945,-2.73013216987657));
#99520=CARTESIAN_POINT('Ctrl Pts',(20.8292063116425,18.9074341615935,-2.73127477248517));
#99521=CARTESIAN_POINT('Ctrl Pts',(20.8250477688962,18.8804227527477,-2.73292614710874));
#99522=CARTESIAN_POINT('Ctrl Pts',(20.8236957219795,18.8719810018652,-2.73344109325815));
#99523=CARTESIAN_POINT('Ctrl Pts',(20.8212342143084,18.8571866076319,-2.73434159695733));
#99524=CARTESIAN_POINT('Ctrl Pts',(20.8201468027287,18.8508304553537,-2.73472784867144));
#99525=CARTESIAN_POINT('Ctrl Pts',(20.8179778700571,18.8384920235643,-2.73547643613149));
#99526=CARTESIAN_POINT('Ctrl Pts',(20.8168995907418,18.8325092451995,-2.73583887075416));
#99527=CARTESIAN_POINT('Ctrl Pts',(20.8142585491144,18.8182087143678,-2.73670392165712));
#99528=CARTESIAN_POINT('Ctrl Pts',(20.8126716421405,18.8098954842522,-2.7372057656217));
#99529=CARTESIAN_POINT('Ctrl Pts',(20.8067544080408,18.7798758001871,-2.73901441726628));
#99530=CARTESIAN_POINT('Ctrl Pts',(20.8021334856037,18.7582275936779,-2.74031196608073));
#99531=CARTESIAN_POINT('Ctrl Pts',(20.755648006654,18.5560379115105,-2.75237780083063));
#99532=CARTESIAN_POINT('Ctrl Pts',(20.6905881497839,18.381659991534,-2.76229230394082));
#99533=CARTESIAN_POINT('Ctrl Pts',(20.5659759708226,18.1470438304773,-2.77677352323143));
#99534=CARTESIAN_POINT('Ctrl Pts',(20.5243020089875,18.0783237933446,-2.78118953506107));
#99535=CARTESIAN_POINT('Ctrl Pts',(20.4584000975061,17.9824094512677,-2.78784585150284));
#99536=CARTESIAN_POINT('Ctrl Pts',(20.4372152844464,17.953205192522,-2.78994414931373));
#99537=CARTESIAN_POINT('Ctrl Pts',(20.410757542257,17.9186266289342,-2.79253521455693));
#99538=CARTESIAN_POINT('Ctrl Pts',(20.4061875651719,17.9127190100488,-2.79298175051942));
#99539=CARTESIAN_POINT('Ctrl Pts',(20.3990238070851,17.9035589777024,-2.79368037788817));
#99540=CARTESIAN_POINT('Ctrl Pts',(20.3964514867217,17.9002897503417,-2.79393096996523));
#99541=CARTESIAN_POINT('Ctrl Pts',(20.3916563357817,17.8942322954638,-2.79439765784973));
#99542=CARTESIAN_POINT('Ctrl Pts',(20.3894360903565,17.8914420947124,-2.79461356985555));
#99543=CARTESIAN_POINT('Ctrl Pts',(20.3843918867449,17.8851357694261,-2.79510370627398));
#99544=CARTESIAN_POINT('Ctrl Pts',(20.3815637505502,17.8816230689712,-2.79537822793867));
#99545=CARTESIAN_POINT('Ctrl Pts',(20.374233244835,17.8725775006318,-2.79608899700515));
#99546=CARTESIAN_POINT('Ctrl Pts',(20.3697141375818,17.8670583565179,-2.79652641012653));
#99547=CARTESIAN_POINT('Ctrl Pts',(20.3418046051799,17.8333219974645,-2.79922262100264));
#99548=CARTESIAN_POINT('Ctrl Pts',(20.3177140423278,17.8056951269798,-2.8015275691923));
#99549=CARTESIAN_POINT('Ctrl Pts',(20.1775031367678,17.6530880782193,-2.8147528921501));
#99550=CARTESIAN_POINT('Ctrl Pts',(20.0473267844066,17.541878455085,-2.82626398317437));
#99551=CARTESIAN_POINT('Ctrl Pts',(19.8257962925328,17.3947515275174,-2.84354582263158));
#99552=CARTESIAN_POINT('Ctrl Pts',(19.7429007297666,17.3474278332049,-2.84960274492326));
#99553=CARTESIAN_POINT('Ctrl Pts',(19.6378408759582,17.2965240889397,-2.85677366252124));
#99554=CARTESIAN_POINT('Ctrl Pts',(19.6184546381155,17.287491125867,-2.85807719036012));
#99555=CARTESIAN_POINT('Ctrl Pts',(19.5907117025869,17.2750725176694,-2.85991542967627));
#99556=CARTESIAN_POINT('Ctrl Pts',(19.5824656181997,17.2714443145796,-2.86045844438309));
#99557=CARTESIAN_POINT('Ctrl Pts',(19.5682063546996,17.2652787073771,-2.86139171707981));
#99558=CARTESIAN_POINT('Ctrl Pts',(19.5622041891893,17.2627162903526,-2.86178282562564));
#99559=CARTESIAN_POINT('Ctrl Pts',(19.5506935440632,17.2578650238011,-2.86252959604228));
#99560=CARTESIAN_POINT('Ctrl Pts',(19.5451870611022,17.2555716241223,-2.86288540976373));
#99561=CARTESIAN_POINT('Ctrl Pts',(19.5308527615449,17.249672488838,-2.86380799082697));
#99562=CARTESIAN_POINT('Ctrl Pts',(19.5220100821921,17.2461030448116,-2.86437352616462));
#99563=CARTESIAN_POINT('Ctrl Pts',(19.4918251342721,17.2341551040104,-2.86629205257813));
#99564=CARTESIAN_POINT('Ctrl Pts',(19.4703705370113,17.226063434367,-2.86763541446476));
#99565=CARTESIAN_POINT('Ctrl Pts',(19.2828153238359,17.1587860275195,-2.8792146453731));
#99566=CARTESIAN_POINT('Ctrl Pts',(19.1100575384729,17.1202183673649,-2.88869114687395));
#99567=CARTESIAN_POINT('Ctrl Pts',(18.8484807130938,17.0953322329895,-2.90299000891541));
#99568=CARTESIAN_POINT('Ctrl Pts',(18.7620438558293,17.0924233279127,-2.90772244744911));
#99569=CARTESIAN_POINT('Ctrl Pts',(18.6380204629066,17.0958413387308,-2.91480728427978));
#99570=CARTESIAN_POINT('Ctrl Pts',(18.6003990385863,17.0978841436868,-2.91699583607903));
#99571=CARTESIAN_POINT('Ctrl Pts',(18.5553165097138,17.1015407302542,-2.91968698448819));
#99572=CARTESIAN_POINT('Ctrl Pts',(18.547781628787,17.1021925373026,-2.92013907789111));
#99573=CARTESIAN_POINT('Ctrl Pts',(18.5360876768861,17.1032672873211,-2.92084452367938));
#99574=CARTESIAN_POINT('Ctrl Pts',(18.5319260058597,17.1036622064947,-2.92109632903089));
#99575=CARTESIAN_POINT('Ctrl Pts',(18.5242185796754,17.1044166388692,-2.92156410733076));
#99576=CARTESIAN_POINT('Ctrl Pts',(18.5206725524296,17.1047727802453,-2.92177988907489));
#99577=CARTESIAN_POINT('Ctrl Pts',(18.5126684751859,17.1055970814703,-2.92226822596466));
#99578=CARTESIAN_POINT('Ctrl Pts',(18.508211028365,17.1060704447268,-2.92254106900114));
#99579=CARTESIAN_POINT('Ctrl Pts',(18.4950898198076,17.1075060226235,-2.92334677932452));
#99580=CARTESIAN_POINT('Ctrl Pts',(18.486430581789,17.1085075828382,-2.92388178153363));
#99581=CARTESIAN_POINT('Ctrl Pts',(18.4248686020642,17.1160136529679,-2.92770748962769));
#99582=CARTESIAN_POINT('Ctrl Pts',(18.3722263723868,17.1244600833069,-2.93109510204498));
#99583=CARTESIAN_POINT('Ctrl Pts',(18.3023671160317,17.1383919761581,-2.93569881183349));
#99584=CARTESIAN_POINT('Ctrl Pts',(18.2848158633758,17.1421248097532,-2.93686471372105));
#99585=CARTESIAN_POINT('Ctrl Pts',(18.2202688798785,17.1567128526648,-2.94118221444833));
#99586=CARTESIAN_POINT('Ctrl Pts',(18.1736014733933,17.1689499012762,-2.94436187204783));
#99587=CARTESIAN_POINT('Ctrl Pts',(18.0226008043547,17.2141113934183,-2.95477312449557));
#99588=CARTESIAN_POINT('Ctrl Pts',(17.9203860230035,17.2535300296179,-2.96200570030163));
#99589=CARTESIAN_POINT('Ctrl Pts',(17.7533808690013,17.3332880376191,-2.97390169377441));
#99590=CARTESIAN_POINT('Ctrl Pts',(17.6868836071066,17.3695425464847,-2.97866449906579));
#99591=CARTESIAN_POINT('Ctrl Pts',(17.6063837415456,17.4192054866225,-2.98445945731136));
#99592=CARTESIAN_POINT('Ctrl Pts',(17.5904362901477,17.429341199235,-2.98560915438306));
#99593=CARTESIAN_POINT('Ctrl Pts',(17.567455419989,17.4443828391994,-2.98726882635567));
#99594=CARTESIAN_POINT('Ctrl Pts',(17.560313071366,17.4491199113118,-2.98778506296745));
#99595=CARTESIAN_POINT('Ctrl Pts',(17.5478447386553,17.4574988394124,-2.98868705568223));
#99596=CARTESIAN_POINT('Ctrl Pts',(17.5425063070238,17.4611218884662,-2.98907351302871));
#99597=CARTESIAN_POINT('Ctrl Pts',(17.5321751884177,17.4682025355165,-2.98982194281896));
#99598=CARTESIAN_POINT('Ctrl Pts',(17.5271806582596,17.4716573202705,-2.99018401675394));
#99599=CARTESIAN_POINT('Ctrl Pts',(17.5152808157448,17.4799645360757,-2.99104732297116));
#99600=CARTESIAN_POINT('Ctrl Pts',(17.5083894844323,17.4848368864155,-2.9915477900786));
#99601=CARTESIAN_POINT('Ctrl Pts',(17.483652863754,17.5025491384645,-2.99334628428657));
#99602=CARTESIAN_POINT('Ctrl Pts',(17.4659783115253,17.5156258942739,-2.99463518982757));
#99603=CARTESIAN_POINT('Ctrl Pts',(17.3000934569141,17.6424036877317,-3.00677956299877));
#99604=CARTESIAN_POINT('Ctrl Pts',(17.1673451492009,17.7749704581813,-3.0167651179066));
#99605=CARTESIAN_POINT('Ctrl Pts',(17.0054418802403,17.9862258147212,-3.03127849372914));
#99606=CARTESIAN_POINT('Ctrl Pts',(16.9607582039768,18.0518638786354,-3.03564441507471));
#99607=CARTESIAN_POINT('Ctrl Pts',(16.9014072497951,18.1505399432923,-3.04223259077679));
#99608=CARTESIAN_POINT('Ctrl Pts',(16.8837303565891,18.1816926485078,-3.04431616260788));
#99609=CARTESIAN_POINT('Ctrl Pts',(16.8633406653445,18.2198500600563,-3.04689088952553));
#99610=CARTESIAN_POINT('Ctrl Pts',(16.8598628487978,18.2264419851936,-3.0473364915599));
#99611=CARTESIAN_POINT('Ctrl Pts',(16.8544998901505,18.2367384266318,-3.04803397273379));
#99612=CARTESIAN_POINT('Ctrl Pts',(16.8525906877086,18.2404304377289,-3.04828436049649));
#99613=CARTESIAN_POINT('Ctrl Pts',(16.8490636419453,18.2473005427728,-3.04875086669966));
#99614=CARTESIAN_POINT('Ctrl Pts',(16.8474429517466,18.2504771107082,-3.0489668025912));
#99615=CARTESIAN_POINT('Ctrl Pts',(16.8437887964376,18.2576842149565,-3.0494572508952));
#99616=CARTESIAN_POINT('Ctrl Pts',(16.8417602029554,18.2617171497949,-3.04973206217267));
#99617=CARTESIAN_POINT('Ctrl Pts',(16.8357860112669,18.273689350793,-3.05054888666941));
#99618=CARTESIAN_POINT('Ctrl Pts',(16.8318774264879,18.2816468329169,-3.05109312190785));
#99619=CARTESIAN_POINT('Ctrl Pts',(16.8031430489102,18.3410877591387,-3.05516696600248));
#99620=CARTESIAN_POINT('Ctrl Pts',(16.7803635666302,18.3935287064521,-3.05880791823012));
#99621=CARTESIAN_POINT('Ctrl Pts',(16.7548404642287,18.4594679460122,-3.0633885546121));
#99622=CARTESIAN_POINT('Ctrl Pts',(16.7500682834686,18.4721578996777,-3.0642702345555));
#99623=CARTESIAN_POINT('Ctrl Pts',(16.7454194666968,18.4848894969994,-3.06515441818778));
#99624=CARTESIAN_POINT('',(16.6200858900717,19.2101715454936,-2.08900427075732));
#99625=CARTESIAN_POINT('Ctrl Pts',(16.747777019274,18.4857290362168,-2.84456321874111));
#99626=CARTESIAN_POINT('Ctrl Pts',(16.8351531090644,18.241375047072,-2.82899806149126));
#99627=CARTESIAN_POINT('Ctrl Pts',(17.3199691688815,17.3916717671322,-2.77104096868093));
#99628=CARTESIAN_POINT('Ctrl Pts',(19.0938031543631,16.7337290395393,-2.67069194031012));
#99629=CARTESIAN_POINT('Ctrl Pts',(21.0117474691636,18.1726377106278,-2.54351613362868));
#99630=CARTESIAN_POINT('Ctrl Pts',(20.8399998558895,20.5641793786163,-2.41634032694726));
#99631=CARTESIAN_POINT('Ctrl Pts',(18.736128084209,21.7142628689015,-2.28916452026583));
#99632=CARTESIAN_POINT('Ctrl Pts',(16.9296978888421,20.7307616435956,-2.18006983762423));
#99633=CARTESIAN_POINT('Ctrl Pts',(16.6216056483476,19.6158003190927,-2.11336709054313));
#99634=CARTESIAN_POINT('Ctrl Pts',(16.6201761352154,19.2101685860996,-2.0890562790225));
#99635=CARTESIAN_POINT('Ctrl Pts',(16.6170001249202,19.210272736479,-2.08722594468162));
#99636=CARTESIAN_POINT('Ctrl Pts',(16.6170670028706,19.0155969299224,-2.07601658232614));
#99637=CARTESIAN_POINT('Ctrl Pts',(16.6439835858641,18.8218627412699,-2.0657352630804));
#99638=CARTESIAN_POINT('Ctrl Pts',(16.7112838353467,18.5840556965883,-2.0521523543399));
#99639=CARTESIAN_POINT('Ctrl Pts',(16.7274347386544,18.5341438219612,-2.04923738527145));
#99640=CARTESIAN_POINT('Ctrl Pts',(16.7454194497489,18.4848895434144,-2.04625067101847));
#99641=CARTESIAN_POINT('Origin',(18.734,19.211,0.));
#99642=CARTESIAN_POINT('',(16.7454193884829,18.484889711202,-1.2445862186816));
#99643=CARTESIAN_POINT('',(16.7454194504776,18.4848895414187,-1.46829793832533));
#99644=CARTESIAN_POINT('',(16.7454194503191,18.4848895418526,0.));
#99645=CARTESIAN_POINT('Ctrl Pts',(16.7454194504776,18.4848895414187,-1.46829793832533));
#99646=CARTESIAN_POINT('Ctrl Pts',(16.6959068598972,18.6204884347014,-1.47674751206437));
#99647=CARTESIAN_POINT('Ctrl Pts',(16.6603893501654,18.7608044574327,-1.48469151238656));
#99648=CARTESIAN_POINT('Ctrl Pts',(16.6244283767766,19.0058873144864,-1.49816090940912));
#99649=CARTESIAN_POINT('Ctrl Pts',(16.6169334230905,19.1090662019796,-1.50372410772867));
#99650=CARTESIAN_POINT('Ctrl Pts',(16.617039406997,19.2724280285841,-1.51286250500369));
#99651=CARTESIAN_POINT('Ctrl Pts',(16.6196337799328,19.332448106488,-1.51629223384452));
#99652=CARTESIAN_POINT('Ctrl Pts',(16.6255428333359,19.4012045822417,-1.52038547531305));
#99653=CARTESIAN_POINT('Ctrl Pts',(16.6263673812465,19.4101334846522,-1.52092023865661));
#99654=CARTESIAN_POINT('Ctrl Pts',(16.6276944043495,19.4235707244116,-1.52173020007817));
#99655=CARTESIAN_POINT('Ctrl Pts',(16.6281546984081,19.4280832559857,-1.52200308581255));
#99656=CARTESIAN_POINT('Ctrl Pts',(16.6290029478587,19.4361424884885,-1.5224920827716));
#99657=CARTESIAN_POINT('Ctrl Pts',(16.6293853698041,19.4396897193852,-1.52270788010183));
#99658=CARTESIAN_POINT('Ctrl Pts',(16.6302310217689,19.4473519268589,-1.52317525487703));
#99659=CARTESIAN_POINT('Ctrl Pts',(16.6306973520588,19.451466458332,-1.52342699932537));
#99660=CARTESIAN_POINT('Ctrl Pts',(16.6320285811027,19.462911980543,-1.52412937420652));
#99661=CARTESIAN_POINT('Ctrl Pts',(16.6329197472504,19.4702397724419,-1.52458144421862));
#99662=CARTESIAN_POINT('Ctrl Pts',(16.6382144776853,19.5119550436418,-1.52716799118256));
#99663=CARTESIAN_POINT('Ctrl Pts',(16.6434236348418,19.546232805256,-1.52934379516798));
#99664=CARTESIAN_POINT('Ctrl Pts',(16.6625928168378,19.6544150201489,-1.53633889055484));
#99665=CARTESIAN_POINT('Ctrl Pts',(16.6796496685526,19.7277085866481,-1.54126750918516));
#99666=CARTESIAN_POINT('Ctrl Pts',(16.7543348629841,19.9855767587457,-1.55897624798418));
#99667=CARTESIAN_POINT('Ctrl Pts',(16.833285513439,20.163028807161,-1.57174489460041));
#99668=CARTESIAN_POINT('Ctrl Pts',(16.9464403129331,20.3453589893003,-1.58492997915281));
#99669=CARTESIAN_POINT('Ctrl Pts',(16.9579092292772,20.3632332997938,-1.58622483245215));
#99670=CARTESIAN_POINT('Ctrl Pts',(16.9742421772088,20.3878647287892,-1.58801295848453));
#99671=CARTESIAN_POINT('Ctrl Pts',(16.9788797317359,20.3947698390144,-1.58851465949724));
#99672=CARTESIAN_POINT('Ctrl Pts',(16.9869555310392,20.4066425543119,-1.58937807984382));
#99673=CARTESIAN_POINT('Ctrl Pts',(16.9903745393692,20.4116230667551,-1.58974052067012));
#99674=CARTESIAN_POINT('Ctrl Pts',(16.9974994140815,20.4219073361421,-1.59048945997367));
#99675=CARTESIAN_POINT('Ctrl Pts',(17.0012083737823,20.4272088813858,-1.59087583543189));
#99676=CARTESIAN_POINT('Ctrl Pts',(17.0099527897475,20.4395868491681,-1.59177868363988));
#99677=CARTESIAN_POINT('Ctrl Pts',(17.0150076272013,20.4466494870373,-1.59229440641937));
#99678=CARTESIAN_POINT('Ctrl Pts',(17.0315678467597,20.4694891907515,-1.59396423982988));
#99679=CARTESIAN_POINT('Ctrl Pts',(17.0432482868361,20.4851385175056,-1.59511156994434));
#99680=CARTESIAN_POINT('Ctrl Pts',(17.1041455565418,20.5644156735477,-1.6009440164131));
#99681=CARTESIAN_POINT('Ctrl Pts',(17.156746131161,20.6253662046906,-1.60549250894985));
#99682=CARTESIAN_POINT('Ctrl Pts',(17.329516928172,20.8039023620081,-1.61926735349304));
#99683=CARTESIAN_POINT('Ctrl Pts',(17.4602834086994,20.9102790533472,-1.62810921921722));
#99684=CARTESIAN_POINT('Ctrl Pts',(17.6034464149036,21.0008434689676,-1.63762169540562));
#99685=CARTESIAN_POINT('Ctrl Pts',(17.6046578327881,21.0016080870819,-1.63770218047912));
#99686=CARTESIAN_POINT('Ctrl Pts',(17.6514439486952,21.0310720037534,-1.64081033113675));
#99687=CARTESIAN_POINT('Ctrl Pts',(17.6980925138912,21.0580203944255,-1.64389965447141));
#99688=CARTESIAN_POINT('Ctrl Pts',(17.7534414804455,21.0872383539285,-1.64761364329193));
#99689=CARTESIAN_POINT('Ctrl Pts',(17.7611948552407,21.0912700644848,-1.64813498479443));
#99690=CARTESIAN_POINT('Ctrl Pts',(17.7729667913062,21.0972991034811,-1.6489285015261));
#99691=CARTESIAN_POINT('Ctrl Pts',(17.7769672159459,21.0993319055185,-1.64919850135907));
#99692=CARTESIAN_POINT('Ctrl Pts',(17.7841567114073,21.1029565087954,-1.64968440566121));
#99693=CARTESIAN_POINT('Ctrl Pts',(17.7873433637962,21.1045529876125,-1.64990001267127));
#99694=CARTESIAN_POINT('Ctrl Pts',(17.7942731517909,21.1080028720176,-1.65036940213231));
#99695=CARTESIAN_POINT('Ctrl Pts',(17.7980176958408,21.109853225316,-1.6506233647053));
#99696=CARTESIAN_POINT('Ctrl Pts',(17.8085430972304,21.115015617342,-1.65133807963303));
#99697=CARTESIAN_POINT('Ctrl Pts',(17.8153361449886,21.1183024583224,-1.65180035323353));
#99698=CARTESIAN_POINT('Ctrl Pts',(17.8558858092826,21.1376556801787,-1.65456508847729));
#99699=CARTESIAN_POINT('Ctrl Pts',(17.8900434268716,21.1528608466435,-1.65691568048034));
#99700=CARTESIAN_POINT('Ctrl Pts',(18.0033889318725,21.1997609526478,-1.66474435179443));
#99701=CARTESIAN_POINT('Ctrl Pts',(18.0840883256608,21.2275752166946,-1.67036021279631));
#99702=CARTESIAN_POINT('Ctrl Pts',(18.3376409819696,21.298161707302,-1.68774741306462));
#99703=CARTESIAN_POINT('Ctrl Pts',(18.5144113666176,21.3240900869336,-1.69943889571769));
#99704=CARTESIAN_POINT('Ctrl Pts',(18.7151610050707,21.3280389542826,-1.71179548129477));
#99705=CARTESIAN_POINT('Ctrl Pts',(18.7379630520414,21.3281190801895,-1.71318717444918));
#99706=CARTESIAN_POINT('Ctrl Pts',(18.7702766298393,21.3277105461314,-1.71514331801955));
#99707=CARTESIAN_POINT('Ctrl Pts',(18.7797897934904,21.3275261230166,-1.71571723815169));
#99708=CARTESIAN_POINT('Ctrl Pts',(18.7952605951424,21.3271218477167,-1.71664745239659));
#99709=CARTESIAN_POINT('Ctrl Pts',(18.80121903906,21.3269409577818,-1.71700496234333));
#99710=CARTESIAN_POINT('Ctrl Pts',(18.8137023079373,21.3265092003526,-1.71775241537211));
#99711=CARTESIAN_POINT('Ctrl Pts',(18.8202269050533,21.3262533079952,-1.71814219699084));
#99712=CARTESIAN_POINT('Ctrl Pts',(18.8357688326794,21.3255717286431,-1.71906861099234));
#99713=CARTESIAN_POINT('Ctrl Pts',(18.8447848767661,21.3251185410959,-1.71960437601916));
#99714=CARTESIAN_POINT('Ctrl Pts',(18.8752584349786,21.3233913204335,-1.72140982091528));
#99715=CARTESIAN_POINT('Ctrl Pts',(18.8966997974882,21.3218481380876,-1.72267106597266));
#99716=CARTESIAN_POINT('Ctrl Pts',(19.0969130637548,21.3043694531506,-1.73437254793194));
#99717=CARTESIAN_POINT('Ctrl Pts',(19.2729982710574,21.2660886617846,-1.74401575230736));
#99718=CARTESIAN_POINT('Ctrl Pts',(19.555684578965,21.1657470774263,-1.76034091505661));
#99719=CARTESIAN_POINT('Ctrl Pts',(19.6655505568961,21.1158377291937,-1.76695024492803));
#99720=CARTESIAN_POINT('Ctrl Pts',(19.778840346635,21.0522191183713,-1.77465072814509));
#99721=CARTESIAN_POINT('Ctrl Pts',(19.787089422591,21.0475135045075,-1.77521680930884));
#99722=CARTESIAN_POINT('Ctrl Pts',(19.7992700049658,21.0404561488919,-1.77606110946159));
#99723=CARTESIAN_POINT('Ctrl Pts',(19.8032261192575,21.0381468165396,-1.77633665612269));
#99724=CARTESIAN_POINT('Ctrl Pts',(19.8102535521807,21.0340140014688,-1.77682854672267));
#99725=CARTESIAN_POINT('Ctrl Pts',(19.8133277818173,21.032195568109,-1.77704456167691));
#99726=CARTESIAN_POINT('Ctrl Pts',(19.8199297122953,21.0282678814746,-1.77751026300074));
#99727=CARTESIAN_POINT('Ctrl Pts',(19.8234558251876,21.0261561633606,-1.77776010497034));
#99728=CARTESIAN_POINT('Ctrl Pts',(19.833177523092,21.0202955018174,-1.77845195410065));
#99729=CARTESIAN_POINT('Ctrl Pts',(19.8393599879735,21.0165250576118,-1.77889533280146));
#99730=CARTESIAN_POINT('Ctrl Pts',(19.8732142644036,20.9956396039212,-1.78134142065681));
#99731=CARTESIAN_POINT('Ctrl Pts',(19.9005064094762,20.9779211028227,-1.78338047178864));
#99732=CARTESIAN_POINT('Ctrl Pts',(20.0617654452043,20.8678645363204,-1.79578646284055));
#99733=CARTESIAN_POINT('Ctrl Pts',(20.1851285139736,20.760963591564,-1.80674330176059));
#99734=CARTESIAN_POINT('Ctrl Pts',(20.3739337424721,20.5548567574695,-1.82500089877527));
#99735=CARTESIAN_POINT('Ctrl Pts',(20.4455824257093,20.4623301204311,-1.83244165709588));
#99736=CARTESIAN_POINT('Ctrl Pts',(20.5170242067805,20.3523666643615,-1.84044863649234));
#99737=CARTESIAN_POINT('Ctrl Pts',(20.52468770223,20.3403054295805,-1.84131661054526));
#99738=CARTESIAN_POINT('Ctrl Pts',(20.5366901839651,20.3209858463645,-1.84269091606629));
#99739=CARTESIAN_POINT('Ctrl Pts',(20.5411087162168,20.3137776609572,-1.84320017559491));
#99740=CARTESIAN_POINT('Ctrl Pts',(20.5488253311113,20.3010182138872,-1.84409555187577));
#99741=CARTESIAN_POINT('Ctrl Pts',(20.5521413978991,20.295478007028,-1.84448232475353));
#99742=CARTESIAN_POINT('Ctrl Pts',(20.5589476627747,20.2839877031702,-1.84528039192358));
#99743=CARTESIAN_POINT('Ctrl Pts',(20.5624342331843,20.278035538149,-1.84569155083534));
#99744=CARTESIAN_POINT('Ctrl Pts',(20.5713090994871,20.262713411274,-1.8467442585542));
#99745=CARTESIAN_POINT('Ctrl Pts',(20.5766548835802,20.2533189593826,-1.84738426606248));
#99746=CARTESIAN_POINT('Ctrl Pts',(20.5986659935689,20.2139389661409,-1.850044925651));
#99747=CARTESIAN_POINT('Ctrl Pts',(20.6146737328174,20.1835905328897,-1.85204204905034));
#99748=CARTESIAN_POINT('Ctrl Pts',(20.6544539887068,20.1035144393947,-1.8571861135451));
#99749=CARTESIAN_POINT('Ctrl Pts',(20.6770353651403,20.0532231073029,-1.8602936657903));
#99750=CARTESIAN_POINT('Ctrl Pts',(20.7384915575997,19.9006805087424,-1.86943806290884));
#99751=CARTESIAN_POINT('Ctrl Pts',(20.7714348766994,19.7962397931314,-1.87532617814154));
#99752=CARTESIAN_POINT('Ctrl Pts',(20.8065009483781,19.6451877511086,-1.8837687736118));
#99753=CARTESIAN_POINT('Ctrl Pts',(20.8153937493393,19.6003314877986,-1.88626856698705));
#99754=CARTESIAN_POINT('Ctrl Pts',(20.8265370763613,19.5327113081147,-1.89006869277782));
#99755=CARTESIAN_POINT('Ctrl Pts',(20.8298827144741,19.5101407308908,-1.89134240181201));
#99756=CARTESIAN_POINT('Ctrl Pts',(20.8330068333032,19.4864279025798,-1.8926900312721));
#99757=CARTESIAN_POINT('Ctrl Pts',(20.8331500026186,19.4853346173429,-1.89275218508388));
#99758=CARTESIAN_POINT('Ctrl Pts',(20.8397581739754,19.4345645203354,-1.89563948799598));
#99759=CARTESIAN_POINT('Ctrl Pts',(20.8444581568153,19.3846781249981,-1.89852074748396));
#99760=CARTESIAN_POINT('Ctrl Pts',(20.8478413750193,19.3268656945797,-1.90195836270283));
#99761=CARTESIAN_POINT('Ctrl Pts',(20.8482551558296,19.3190525321089,-1.90242502334476));
#99762=CARTESIAN_POINT('Ctrl Pts',(20.8488465800877,19.3065757422154,-1.90317380144847));
#99763=CARTESIAN_POINT('Ctrl Pts',(20.849052133623,19.3019134253639,-1.90345439982381));
#99764=CARTESIAN_POINT('Ctrl Pts',(20.8493885683665,19.2936625649046,-1.9039524395378));
#99765=CARTESIAN_POINT('Ctrl Pts',(20.8495257375652,19.2900743217089,-1.90416952603827));
#99766=CARTESIAN_POINT('Ctrl Pts',(20.849796819096,19.2824766611927,-1.90463024391723));
#99767=CARTESIAN_POINT('Ctrl Pts',(20.8499284627948,19.2784672699049,-1.90487399344614));
#99768=CARTESIAN_POINT('Ctrl Pts',(20.8502524268373,19.2676644023794,-1.9055323819951));
#99769=CARTESIAN_POINT('Ctrl Pts',(20.8504234285035,19.2608704017992,-1.90594818576546));
#99770=CARTESIAN_POINT('Ctrl Pts',(20.8511046952856,19.2273958503391,-1.90800505444492));
#99771=CARTESIAN_POINT('Ctrl Pts',(20.8511431376046,19.2007094233868,-1.90967037746517));
#99772=CARTESIAN_POINT('Ctrl Pts',(20.8498011711394,19.1238747345776,-1.9145252321067));
#99773=CARTESIAN_POINT('Ctrl Pts',(20.8471427593648,19.0737687499926,-1.91776473227241));
#99774=CARTESIAN_POINT('Ctrl Pts',(20.8311335823854,18.8934261565449,-1.92958818445611));
#99775=CARTESIAN_POINT('Ctrl Pts',(20.8074923777699,18.7643968725743,-1.93833645646128));
#99776=CARTESIAN_POINT('Ctrl Pts',(20.7435780671029,18.5369145299891,-1.95370070928406));
#99777=CARTESIAN_POINT('Ctrl Pts',(20.7075330014761,18.4377157463494,-1.96038329006193));
#99778=CARTESIAN_POINT('Ctrl Pts',(20.6584568122342,18.3287565869069,-1.96767812183041));
#99779=CARTESIAN_POINT('Ctrl Pts',(20.6525431892436,18.3159695490272,-1.96853368315175));
#99780=CARTESIAN_POINT('Ctrl Pts',(20.6429021319407,18.2956573636174,-1.96989210251203));
#99781=CARTESIAN_POINT('Ctrl Pts',(20.6392568829303,18.288093880979,-1.97039778420121));
#99782=CARTESIAN_POINT('Ctrl Pts',(20.6327330440303,18.2747610376537,-1.97128900800427));
#99783=CARTESIAN_POINT('Ctrl Pts',(20.6298729306371,18.268982803017,-1.97167518707565));
#99784=CARTESIAN_POINT('Ctrl Pts',(20.6238872568839,18.2570277380775,-1.97247409306763));
#99785=CARTESIAN_POINT('Ctrl Pts',(20.6207577032444,18.2508529845656,-1.97288667440835));
#99786=CARTESIAN_POINT('Ctrl Pts',(20.6126136484626,18.2349779733188,-1.97394733597398));
#99787=CARTESIAN_POINT('Ctrl Pts',(20.6075542423733,18.2253008854613,-1.97459382895316));
#99788=CARTESIAN_POINT('Ctrl Pts',(20.5858312234504,18.1845230029864,-1.97731826079207));
#99789=CARTESIAN_POINT('Ctrl Pts',(20.5684657742618,18.1538011341689,-1.97937120721142));
#99790=CARTESIAN_POINT('Ctrl Pts',(20.5209125952416,18.0743760146279,-1.98469258930912));
#99791=CARTESIAN_POINT('Ctrl Pts',(20.4895012530008,18.0264381528055,-1.98791797766205));
#99792=CARTESIAN_POINT('Ctrl Pts',(20.3658038554172,17.853407971902,-1.99972432972039));
#99793=CARTESIAN_POINT('Ctrl Pts',(20.2617863034488,17.737329348791,-2.00794636938961));
#99794=CARTESIAN_POINT('Ctrl Pts',(20.1334485206014,17.6224418669102,-2.01751895948848));
#99795=CARTESIAN_POINT('Ctrl Pts',(20.1207564696309,17.6113501705525,-2.01846062217564));
#99796=CARTESIAN_POINT('Ctrl Pts',(20.0673758786275,17.5658131618407,-2.02240670428345));
#99797=CARTESIAN_POINT('Ctrl Pts',(20.025529327739,17.532762250327,-2.02546577719365));
#99798=CARTESIAN_POINT('Ctrl Pts',(19.9754439900595,17.4961875274164,-2.02914613715852));
#99799=CARTESIAN_POINT('Ctrl Pts',(19.9683721763111,17.4910900253156,-2.02966621520578));
#99800=CARTESIAN_POINT('Ctrl Pts',(19.957616671921,17.4834377480025,-2.03045818028469));
#99801=CARTESIAN_POINT('Ctrl Pts',(19.9539559186703,17.4808506856397,-2.03072790456617));
#99802=CARTESIAN_POINT('Ctrl Pts',(19.9473699942445,17.4762276925308,-2.03121351427578));
#99803=CARTESIAN_POINT('Ctrl Pts',(19.9444478764161,17.4741875058379,-2.03142910380594));
#99804=CARTESIAN_POINT('Ctrl Pts',(19.9380869924229,17.4697702651024,-2.03189869131741));
#99805=CARTESIAN_POINT('Ctrl Pts',(19.9346463782718,17.467396045927,-2.03215287070863));
#99806=CARTESIAN_POINT('Ctrl Pts',(19.9249615556566,17.4607552264595,-2.03286879681091));
#99807=CARTESIAN_POINT('Ctrl Pts',(19.9187015568244,17.4565119231947,-2.03333207289827));
#99808=CARTESIAN_POINT('Ctrl Pts',(19.8811282478524,17.4313358486846,-2.03611516891385));
#99809=CARTESIAN_POINT('Ctrl Pts',(19.8492856113889,17.4112096487811,-2.03848385080122));
#99810=CARTESIAN_POINT('Ctrl Pts',(19.742700406754,17.3477570119258,-2.04640234122446));
#99811=CARTESIAN_POINT('Ctrl Pts',(19.6658448826362,17.3081562971225,-2.05209315702692));
#99812=CARTESIAN_POINT('Ctrl Pts',(19.4253935060272,17.2023290232827,-2.06944986560032));
#99813=CARTESIAN_POINT('Ctrl Pts',(19.2557187035422,17.1517240442912,-2.08103081022248));
#99814=CARTESIAN_POINT('Ctrl Pts',(19.0590957549896,17.1189848744022,-2.09329913705833));
#99815=CARTESIAN_POINT('Ctrl Pts',(19.0364221906489,17.1155870528465,-2.09469854304351));
#99816=CARTESIAN_POINT('Ctrl Pts',(19.0042455743057,17.1112982950912,-2.09666353364091));
#99817=CARTESIAN_POINT('Ctrl Pts',(18.9947854407372,17.1101023636118,-2.09723870471809));
#99818=CARTESIAN_POINT('Ctrl Pts',(18.9793947879915,17.1082622662116,-2.09817039109011));
#99819=CARTESIAN_POINT('Ctrl Pts',(18.9734691360716,17.1075791878296,-2.0985281298787));
#99820=CARTESIAN_POINT('Ctrl Pts',(18.9610542218372,17.1062012038786,-2.09927562112541));
#99821=CARTESIAN_POINT('Ctrl Pts',(18.9545644652573,17.1055112420284,-2.09966521405193));
#99822=CARTESIAN_POINT('Ctrl Pts',(18.9391085242532,17.103940281024,-2.10059037847836));
#99823=CARTESIAN_POINT('Ctrl Pts',(18.9301396558038,17.1030864805939,-2.1011250888805));
#99824=CARTESIAN_POINT('Ctrl Pts',(18.8998610642644,17.1003990045108,-2.10292320890595));
#99825=CARTESIAN_POINT('Ctrl Pts',(18.8785286466909,17.0988309787259,-2.10417827801084));
#99826=CARTESIAN_POINT('Ctrl Pts',(18.6920726549447,17.0879638122336,-2.11505404151969));
#99827=CARTESIAN_POINT('Ctrl Pts',(18.526409712385,17.09771951267,-2.12401221140242));
#99828=CARTESIAN_POINT('Ctrl Pts',(18.3016027589193,17.1376739193637,-2.13641574453864));
#99829=CARTESIAN_POINT('Ctrl Pts',(18.2401735316896,17.1514409959104,-2.13983910272743));
#99830=CARTESIAN_POINT('Ctrl Pts',(18.1596221228129,17.1733049278557,-2.14447025566488));
#99831=CARTESIAN_POINT('Ctrl Pts',(18.1398730572307,17.178975322293,-2.14561733047005));
#99832=CARTESIAN_POINT('Ctrl Pts',(18.0701940452841,17.2000843253544,-2.14971557967471));
#99833=CARTESIAN_POINT('Ctrl Pts',(18.0207605181586,17.2170820795169,-2.1527166975314));
#99834=CARTESIAN_POINT('Ctrl Pts',(17.963919663373,17.2390110321689,-2.15633246707259));
#99835=CARTESIAN_POINT('Ctrl Pts',(17.9558477430367,17.2421822650977,-2.15684989471024));
#99836=CARTESIAN_POINT('Ctrl Pts',(17.9436426265262,17.2470640973833,-2.15763860723274));
#99837=CARTESIAN_POINT('Ctrl Pts',(17.9394948791528,17.2487383916779,-2.15790775585106));
#99838=CARTESIAN_POINT('Ctrl Pts',(17.9320524889223,17.2517700781387,-2.15839275424732));
#99839=CARTESIAN_POINT('Ctrl Pts',(17.9287559423977,17.2531226533227,-2.15860831140802));
#99840=CARTESIAN_POINT('Ctrl Pts',(17.9215924346766,17.2560829977624,-2.15907832761102));
#99841=CARTESIAN_POINT('Ctrl Pts',(17.9177268745272,17.257693899625,-2.15933297079279));
#99842=CARTESIAN_POINT('Ctrl Pts',(17.9070029859586,17.2622002772095,-2.16004217280865));
#99843=CARTESIAN_POINT('Ctrl Pts',(17.9001551904168,17.2651204429536,-2.16049818997774));
#99844=CARTESIAN_POINT('Ctrl Pts',(17.8601330465235,17.2824374889262,-2.16318129240295));
#99845=CARTESIAN_POINT('Ctrl Pts',(17.8273186912187,17.2976454969852,-2.16545337888392));
#99846=CARTESIAN_POINT('Ctrl Pts',(17.7224518637009,17.3495499852349,-2.17291349038553));
#99847=CARTESIAN_POINT('Ctrl Pts',(17.6521101730921,17.389533982468,-2.17822661167641));
#99848=CARTESIAN_POINT('Ctrl Pts',(17.4293354433018,17.5336298415982,-2.19574502878615));
#99849=CARTESIAN_POINT('Ctrl Pts',(17.2881636943055,17.653660993577,-2.2078955885692));
#99850=CARTESIAN_POINT('Ctrl Pts',(17.1494254195771,17.8069679861631,-2.22061254355502));
#99851=CARTESIAN_POINT('Ctrl Pts',(17.1347790983335,17.8236734113778,-2.22196799819656));
#99852=CARTESIAN_POINT('Ctrl Pts',(17.1149114023867,17.8470671016292,-2.22382550562645));
#99853=CARTESIAN_POINT('Ctrl Pts',(17.1094636043675,17.853560373087,-2.2243368652928));
#99854=CARTESIAN_POINT('Ctrl Pts',(17.1001735352377,17.8647693069741,-2.22521244387439));
#99855=CARTESIAN_POINT('Ctrl Pts',(17.0963123530989,17.8694690953277,-2.22557743192844));
#99856=CARTESIAN_POINT('Ctrl Pts',(17.0884005770431,17.8791842848849,-2.22632757160391));
#99857=CARTESIAN_POINT('Ctrl Pts',(17.084352526464,17.88420168287,-2.22671261802951));
#99858=CARTESIAN_POINT('Ctrl Pts',(17.0749966718327,17.8959069027328,-2.22760547801569));
#99859=CARTESIAN_POINT('Ctrl Pts',(17.0697062578163,17.9026085294009,-2.22811259110002));
#99860=CARTESIAN_POINT('Ctrl Pts',(17.0529469528597,17.9241044909288,-2.22972639706376));
#99861=CARTESIAN_POINT('Ctrl Pts',(17.0416334768823,17.9390192677116,-2.23082693703694));
#99862=CARTESIAN_POINT('Ctrl Pts',(16.9927534729308,18.0052655857988,-2.2356344357632));
#99863=CARTESIAN_POINT('Ctrl Pts',(16.957311731321,18.0581275742994,-2.23925948062348));
#99864=CARTESIAN_POINT('Ctrl Pts',(16.8873536190559,18.1733794162606,-2.24680663626997));
#99865=CARTESIAN_POINT('Ctrl Pts',(16.8534986323758,18.236077063811,-2.25070731916699));
#99866=CARTESIAN_POINT('Ctrl Pts',(16.7941561418751,18.3606179444794,-2.25821639434393));
#99867=CARTESIAN_POINT('Ctrl Pts',(16.7683116637394,18.4221952095568,-2.26182386230899));
#99868=CARTESIAN_POINT('Ctrl Pts',(16.7454194503191,18.4848895418526,-2.26547384646965));
#99869=CARTESIAN_POINT('Ctrl Pts',(16.7454194497489,18.4848895434144,-2.04625067101847));
#99870=CARTESIAN_POINT('Ctrl Pts',(16.748932204389,18.475269250122,-2.04566730916763));
#99871=CARTESIAN_POINT('Ctrl Pts',(16.7525149174804,18.4656740442466,-2.04508120036617));
#99872=CARTESIAN_POINT('Ctrl Pts',(16.7671937061732,18.4272154823377,-2.04271340093804));
#99873=CARTESIAN_POINT('Ctrl Pts',(16.7788510679927,18.3985730221787,-2.04090763423702));
#99874=CARTESIAN_POINT('Ctrl Pts',(16.7939618142308,18.3636561223643,-2.03864174979379));
#99875=CARTESIAN_POINT('Ctrl Pts',(16.7968258179881,18.3571288185766,-2.03821535470679));
#99876=CARTESIAN_POINT('Ctrl Pts',(16.8013829450996,18.3468836841518,-2.03754146625148));
#99877=CARTESIAN_POINT('Ctrl Pts',(16.8030539896864,18.343156008944,-2.03729530481808));
#99878=CARTESIAN_POINT('Ctrl Pts',(16.8062079246755,18.3361745887211,-2.03683241795746));
#99879=CARTESIAN_POINT('Ctrl Pts',(16.8076882727687,18.3329197560843,-2.03661584871557));
#99880=CARTESIAN_POINT('Ctrl Pts',(16.8111000197742,18.3254685176877,-2.03611831500188));
#99881=CARTESIAN_POINT('Ctrl Pts',(16.813036907477,18.3212746848889,-2.03583701564578));
#99882=CARTESIAN_POINT('Ctrl Pts',(16.8190812869896,18.3082988768954,-2.03496280912999));
#99883=CARTESIAN_POINT('Ctrl Pts',(16.823235323755,18.2995388988545,-2.03436713610167));
#99884=CARTESIAN_POINT('Ctrl Pts',(16.8705008587748,18.2016091896507,-2.02764871579488));
#99885=CARTESIAN_POINT('Ctrl Pts',(16.9197543466835,18.1155517304313,-2.02119661547279));
#99886=CARTESIAN_POINT('Ctrl Pts',(17.0685235620562,17.8933376474788,-2.00358053880378));
#99887=CARTESIAN_POINT('Ctrl Pts',(17.1785843751989,17.7650591625204,-1.99239369273905));
#99888=CARTESIAN_POINT('Ctrl Pts',(17.3255714047026,17.6301831975143,-1.97986683303894));
#99889=CARTESIAN_POINT('Ctrl Pts',(17.3489064487713,17.6096977540831,-1.97793714026745));
#99890=CARTESIAN_POINT('Ctrl Pts',(17.3842834551674,17.5799930623691,-1.97509721056029));
#99891=CARTESIAN_POINT('Ctrl Pts',(17.3959866756151,17.5703785493105,-1.97417113595211));
#99892=CARTESIAN_POINT('Ctrl Pts',(17.4148938305261,17.5551827028855,-1.97269609917014));
#99893=CARTESIAN_POINT('Ctrl Pts',(17.4220322072816,17.5495209833677,-1.97214392183847));
#99894=CARTESIAN_POINT('Ctrl Pts',(17.4357163011011,17.5388107870854,-1.97109429581479));
#99895=CARTESIAN_POINT('Ctrl Pts',(17.4422554552983,17.5337542336096,-1.97059653054046));
#99896=CARTESIAN_POINT('Ctrl Pts',(17.4537845048468,17.5249465454373,-1.96972553507797));
#99897=CARTESIAN_POINT('Ctrl Pts',(17.4587616553858,17.5211789646849,-1.96935165785627));
#99898=CARTESIAN_POINT('Ctrl Pts',(17.4686169661866,17.5137870764052,-1.96861550761198));
#99899=CARTESIAN_POINT('Ctrl Pts',(17.4734942099634,17.5101616523759,-1.96825319301647));
#99900=CARTESIAN_POINT('Ctrl Pts',(17.4851946312962,17.5015422952822,-1.96738872132745));
#99901=CARTESIAN_POINT('Ctrl Pts',(17.492032283288,17.4965681154039,-1.96688733417987));
#99902=CARTESIAN_POINT('Ctrl Pts',(17.5168356703837,17.478750681511,-1.96508206434312));
#99903=CARTESIAN_POINT('Ctrl Pts',(17.5349726937722,17.4661474905479,-1.9637873946628));
#99904=CARTESIAN_POINT('Ctrl Pts',(17.7074868914954,17.3502299601347,-1.95169903557469));
#99905=CARTESIAN_POINT('Ctrl Pts',(17.8746285822612,17.2673742462143,-1.94176382026612));
#99906=CARTESIAN_POINT('Ctrl Pts',(18.1261998595004,17.1815483970631,-1.92727297071972));
#99907=CARTESIAN_POINT('Ctrl Pts',(18.2033482274414,17.1600242529721,-1.9228711878646));
#99908=CARTESIAN_POINT('Ctrl Pts',(18.3166925849788,17.1352255324177,-1.91623421921975));
#99909=CARTESIAN_POINT('Ctrl Pts',(18.3520505310455,17.1284296232213,-1.91414009170023));
#99910=CARTESIAN_POINT('Ctrl Pts',(18.3949259879772,17.1213173605547,-1.91155365263428));
#99911=CARTESIAN_POINT('Ctrl Pts',(18.4022961761574,17.1201347990098,-1.91110737977979));
#99912=CARTESIAN_POINT('Ctrl Pts',(18.4137821978192,17.1183541016037,-1.91040907501757));
#99913=CARTESIAN_POINT('Ctrl Pts',(18.417893884448,17.1177290619857,-1.9101585401916));
#99914=CARTESIAN_POINT('Ctrl Pts',(18.4255343849237,17.1165906129626,-1.90969190132036));
#99915=CARTESIAN_POINT('Ctrl Pts',(18.4290626637494,17.1160740021307,-1.90947598071486));
#99916=CARTESIAN_POINT('Ctrl Pts',(18.4370573984633,17.1149240372454,-1.9089857507221));
#99917=CARTESIAN_POINT('Ctrl Pts',(18.4415245611604,17.1142960468752,-1.90871114361393));
#99918=CARTESIAN_POINT('Ctrl Pts',(18.4530650521396,17.1127112918473,-1.90800001530098));
#99919=CARTESIAN_POINT('Ctrl Pts',(18.4601412069207,17.1117760229477,-1.90756232648785));
#99920=CARTESIAN_POINT('Ctrl Pts',(18.503651265195,17.1062489510007,-1.90486145973869));
#99921=CARTESIAN_POINT('Ctrl Pts',(18.540192475817,17.1025703031983,-1.90255195330837));
#99922=CARTESIAN_POINT('Ctrl Pts',(18.7466635844147,17.0871969396967,-1.88933835460756));
#99923=CARTESIAN_POINT('Ctrl Pts',(18.9174228130529,17.0950938248628,-1.87784603500694));
#99924=CARTESIAN_POINT('Ctrl Pts',(19.1795617803202,17.1392175761917,-1.8605700067175));
#99925=CARTESIAN_POINT('Ctrl Pts',(19.2725582170084,17.1614227207803,-1.85450263010928));
#99926=CARTESIAN_POINT('Ctrl Pts',(19.3841840461219,17.1962027757636,-1.84732074178399));
#99927=CARTESIAN_POINT('Ctrl Pts',(19.4045223051533,17.2028797247869,-1.84601605000661));
#99928=CARTESIAN_POINT('Ctrl Pts',(19.4332751879296,17.2128047072667,-1.84417646600841));
#99929=CARTESIAN_POINT('Ctrl Pts',(19.4417752063122,17.2157996397327,-1.84363325417258));
#99930=CARTESIAN_POINT('Ctrl Pts',(19.4563978256583,17.2210570408857,-1.84269974620621));
#99931=CARTESIAN_POINT('Ctrl Pts',(19.4625295138347,17.2232936967456,-1.84230859842226));
#99932=CARTESIAN_POINT('Ctrl Pts',(19.474244484527,17.2276284573484,-1.84156182335729));
#99933=CARTESIAN_POINT('Ctrl Pts',(19.4798294267272,17.2297218669703,-1.84120604388603));
#99934=CARTESIAN_POINT('Ctrl Pts',(19.4943170475591,17.2352222164258,-1.84028370318293));
#99935=CARTESIAN_POINT('Ctrl Pts',(19.5032057587659,17.2386657565024,-1.83971837262315));
#99936=CARTESIAN_POINT('Ctrl Pts',(19.5333738497084,17.2505880191995,-1.83780131862885));
#99937=CARTESIAN_POINT('Ctrl Pts',(19.5545392176772,17.2593521991455,-1.8364592038496));
#99938=CARTESIAN_POINT('Ctrl Pts',(19.7376080157621,17.3386622950578,-1.82486499101896));
#99939=CARTESIAN_POINT('Ctrl Pts',(19.8902343827304,17.4288646997646,-1.81537503189025));
#99940=CARTESIAN_POINT('Ctrl Pts',(20.0980772799964,17.5897608909292,-1.8010709118068));
#99941=CARTESIAN_POINT('Ctrl Pts',(20.1629633828687,17.6466520925966,-1.79634831694525));
#99942=CARTESIAN_POINT('Ctrl Pts',(20.2509187011146,17.733819496642,-1.78927676085419));
#99943=CARTESIAN_POINT('Ctrl Pts',(20.2769298804605,17.7610098014468,-1.78709094393442));
#99944=CARTESIAN_POINT('Ctrl Pts',(20.3072797335607,17.7944771309119,-1.78440282599807));
#99945=CARTESIAN_POINT('Ctrl Pts',(20.31232836727,17.8001046389454,-1.78395089556875));
#99946=CARTESIAN_POINT('Ctrl Pts',(20.3201211746591,17.8088851366176,-1.7832456490346));
#99947=CARTESIAN_POINT('Ctrl Pts',(20.3228863945706,17.812019480023,-1.7829938785437));
#99948=CARTESIAN_POINT('Ctrl Pts',(20.3279921801586,17.8178414909012,-1.78252613341434));
#99949=CARTESIAN_POINT('Ctrl Pts',(20.3303352480225,17.8205268872724,-1.78231034977703));
#99950=CARTESIAN_POINT('Ctrl Pts',(20.3356104915107,17.8266037658478,-1.78182196699511));
#99951=CARTESIAN_POINT('Ctrl Pts',(20.338538664505,17.829998633996,-1.78154907971064));
#99952=CARTESIAN_POINT('Ctrl Pts',(20.3471307456788,17.8400243453229,-1.78074310876765));
#99953=CARTESIAN_POINT('Ctrl Pts',(20.3527644107552,17.8466808200299,-1.78020788809811));
#99954=CARTESIAN_POINT('Ctrl Pts',(20.3925763987801,17.8943145297086,-1.77637830335595));
#99955=CARTESIAN_POINT('Ctrl Pts',(20.4252329226406,17.9365328710557,-1.77298682021617));
#99956=CARTESIAN_POINT('Ctrl Pts',(20.4665200388632,17.9942934607574,-1.76839814780399));
#99957=CARTESIAN_POINT('Ctrl Pts',(20.4766030344262,18.0087790853131,-1.76725143660039));
#99958=CARTESIAN_POINT('Ctrl Pts',(20.5136858735944,18.063500534582,-1.76293908919992));
#99959=CARTESIAN_POINT('Ctrl Pts',(20.5394824044578,18.1045327018757,-1.75974481577322));
#99960=CARTESIAN_POINT('Ctrl Pts',(20.6188535677183,18.2409584592925,-1.7493186861675));
#99961=CARTESIAN_POINT('Ctrl Pts',(20.6664533521603,18.339632643482,-1.74208588986972));
#99962=CARTESIAN_POINT('Ctrl Pts',(20.7262430089122,18.492882337104,-1.73151223758427));
#99963=CARTESIAN_POINT('Ctrl Pts',(20.7442598257454,18.5449809023694,-1.72802300248184));
#99964=CARTESIAN_POINT('Ctrl Pts',(20.7701617750288,18.6305596757276,-1.7224653029267));
#99965=CARTESIAN_POINT('Ctrl Pts',(20.7793001331969,18.6636305401208,-1.72035839656378));
#99966=CARTESIAN_POINT('Ctrl Pts',(20.790255861212,18.707395339042,-1.71762183079164));
#99967=CARTESIAN_POINT('Ctrl Pts',(20.7928002593873,18.7179002940177,-1.71696882869671));
#99968=CARTESIAN_POINT('Ctrl Pts',(20.7968365313947,18.7351407496521,-1.71590333646862));
#99969=CARTESIAN_POINT('Ctrl Pts',(20.7983761102126,18.7418647756417,-1.71548931686118));
#99970=CARTESIAN_POINT('Ctrl Pts',(20.8012930921926,18.7548969865183,-1.71468981394894));
#99971=CARTESIAN_POINT('Ctrl Pts',(20.8026745529531,18.7612041759596,-1.71430420428969));
#99972=CARTESIAN_POINT('Ctrl Pts',(20.8057982328307,18.775784467652,-1.71341580430024));
#99973=CARTESIAN_POINT('Ctrl Pts',(20.8075197986331,18.784061919013,-1.71291367999694));
#99974=CARTESIAN_POINT('Ctrl Pts',(20.8120175446899,18.8063566176257,-1.71156711398095));
#99975=CARTESIAN_POINT('Ctrl Pts',(20.814701499101,18.820392179435,-1.71072561347498));
#99976=CARTESIAN_POINT('Ctrl Pts',(20.8380194479748,18.949398917796,-1.70304550623693));
#99977=CARTESIAN_POINT('Ctrl Pts',(20.8492485377539,19.0658729944758,-1.69652341872511));
#99978=CARTESIAN_POINT('Ctrl Pts',(20.8529860109224,19.3453574992842,-1.68122168989833));
#99979=CARTESIAN_POINT('Ctrl Pts',(20.8364044404087,19.5077109611391,-1.67262493106746));
#99980=CARTESIAN_POINT('Ctrl Pts',(20.7943952495572,19.6983622548763,-1.66141634795089));
#99981=CARTESIAN_POINT('Ctrl Pts',(20.7866510683782,19.7300124087444,-1.65951615396292));
#99982=CARTESIAN_POINT('Ctrl Pts',(20.7762964353091,19.7684645758903,-1.65714514399646));
#99983=CARTESIAN_POINT('Ctrl Pts',(20.7743768275969,19.7754500695405,-1.65671186732123));
#99984=CARTESIAN_POINT('Ctrl Pts',(20.7713118568887,19.786383607601,-1.65602952419425));
#99985=CARTESIAN_POINT('Ctrl Pts',(20.7701907632999,19.7903384787037,-1.65578184594555));
#99986=CARTESIAN_POINT('Ctrl Pts',(20.7680740637434,19.7977234957114,-1.65531769627363));
#99987=CARTESIAN_POINT('Ctrl Pts',(20.7670812934255,19.8011543958,-1.65510139062656));
#99988=CARTESIAN_POINT('Ctrl Pts',(20.764795734403,19.8089788118065,-1.65460656181675));
#99989=CARTESIAN_POINT('Ctrl Pts',(20.7634973726848,19.8133706397177,-1.65432771735529));
#99990=CARTESIAN_POINT('Ctrl Pts',(20.7594643792966,19.8268515555118,-1.65346848953093));
#99991=CARTESIAN_POINT('Ctrl Pts',(20.7566829071503,19.8359263473696,-1.65288547246445));
#99992=CARTESIAN_POINT('Ctrl Pts',(20.73123563527,19.9170003172269,-1.64763729051895));
#99993=CARTESIAN_POINT('Ctrl Pts',(20.7047974379205,19.9877506534473,-1.64277918045029));
#99994=CARTESIAN_POINT('Ctrl Pts',(20.6205212509165,20.1810880772827,-1.62898763264374));
#99995=CARTESIAN_POINT('Ctrl Pts',(20.5546053160047,20.2997760414597,-1.61993439762496));
#99996=CARTESIAN_POINT('Ctrl Pts',(20.4268030116346,20.4854398131255,-1.60532705951748));
#99997=CARTESIAN_POINT('Ctrl Pts',(20.3711298320927,20.5562094215129,-1.59962720805163));
#99998=CARTESIAN_POINT('Ctrl Pts',(20.2972855535347,20.6386754208425,-1.59283220891481));
#99999=CARTESIAN_POINT('Ctrl Pts',(20.2832287132102,20.6539169315409,-1.5915690577714));
#100000=CARTESIAN_POINT('Ctrl Pts',(20.2628224254177,20.6754009534606,-1.58977744489934));
#100001=CARTESIAN_POINT('Ctrl Pts',(20.2566543319473,20.6818133634611,-1.58924124211741));
#100002=CARTESIAN_POINT('Ctrl Pts',(20.2459060944276,20.6928472565524,-1.58831598730404));
#100003=CARTESIAN_POINT('Ctrl Pts',(20.2413447683426,20.6974868250126,-1.58792612317244));
#100004=CARTESIAN_POINT('Ctrl Pts',(20.2325437552783,20.7063566402202,-1.58717919149632));
#100005=CARTESIAN_POINT('Ctrl Pts',(20.2283073700397,20.7105900616215,-1.5868219842864));
#100006=CARTESIAN_POINT('Ctrl Pts',(20.2171856920302,20.7216100308647,-1.58589023947696));
#100007=CARTESIAN_POINT('Ctrl Pts',(20.2102717259589,20.7283675422379,-1.58531698364121));
#100008=CARTESIAN_POINT('Ctrl Pts',(20.1862330012043,20.7515424639579,-1.58334411275167));
#100009=CARTESIAN_POINT('Ctrl Pts',(20.1688783514593,20.7677196139166,-1.58195489215878));
#100010=CARTESIAN_POINT('Ctrl Pts',(20.0307366418845,20.8922151955322,-1.57115672235753));
#100011=CARTESIAN_POINT('Ctrl Pts',(19.8981324675179,20.9866162411614,-1.56237404407504));
#100012=CARTESIAN_POINT('Ctrl Pts',(19.6418803015186,21.1278811990845,-1.54647761837973));
#100013=CARTESIAN_POINT('Ctrl Pts',(19.522174520254,21.1801244835777,-1.53938848268958));
#100014=CARTESIAN_POINT('Ctrl Pts',(19.3871558879411,21.2247571373537,-1.53099654831876));
#100015=CARTESIAN_POINT('Ctrl Pts',(19.3758337498979,21.2283943206682,-1.53028982671437));
#100016=CARTESIAN_POINT('Ctrl Pts',(19.3596897455559,21.2334308496959,-1.52927706824115));
#100017=CARTESIAN_POINT('Ctrl Pts',(19.354892380384,21.2349088048366,-1.52897548389518));
#100018=CARTESIAN_POINT('Ctrl Pts',(19.3466139729639,21.2374269835953,-1.52845390420199));
#100019=CARTESIAN_POINT('Ctrl Pts',(19.3431353897502,21.2384753454774,-1.52823438350641));
#100020=CARTESIAN_POINT('Ctrl Pts',(19.3363837941764,21.240491170953,-1.52780760386014));
#100021=CARTESIAN_POINT('Ctrl Pts',(19.3331111342183,21.2414596762644,-1.52760041314822));
#100022=CARTESIAN_POINT('Ctrl Pts',(19.3242717952368,21.2440523440794,-1.52703996155802));
#100023=CARTESIAN_POINT('Ctrl Pts',(19.3187008095448,21.2456615412687,-1.52668584307665));
#100024=CARTESIAN_POINT('Ctrl Pts',(19.2979796640321,21.2515547824242,-1.5253655730213));
#100025=CARTESIAN_POINT('Ctrl Pts',(19.2827889003846,21.2556925418607,-1.52439146539274));
#100026=CARTESIAN_POINT('Ctrl Pts',(19.1401759622143,21.2928347129148,-1.51519755641148));
#100027=CARTESIAN_POINT('Ctrl Pts',(19.00999319318,21.3140540483049,-1.50645963863266));
#100028=CARTESIAN_POINT('Ctrl Pts',(18.7197366709189,21.333939608509,-1.48724143405048));
#100029=CARTESIAN_POINT('Ctrl Pts',(18.5600264604325,21.3268514654846,-1.47686840382037));
#100030=CARTESIAN_POINT('Ctrl Pts',(18.3815830274096,21.2985689560941,-1.46577185151761));
#100031=CARTESIAN_POINT('Ctrl Pts',(18.3606155230474,21.2949208126232,-1.46447480700474));
#100032=CARTESIAN_POINT('Ctrl Pts',(18.330871935262,21.2892823696761,-1.46264402259855));
#100033=CARTESIAN_POINT('Ctrl Pts',(18.3220485519764,21.2875514327981,-1.46210207166813));
#100034=CARTESIAN_POINT('Ctrl Pts',(18.3068431988327,21.2844677766219,-1.46117003497377));
#100035=CARTESIAN_POINT('Ctrl Pts',(18.3004560133068,21.2831416859263,-1.46077910482167));
#100036=CARTESIAN_POINT('Ctrl Pts',(18.2882362799637,21.2805456832788,-1.46003227186534));
#100037=CARTESIAN_POINT('Ctrl Pts',(18.2824027834691,21.2792805864833,-1.45967621914014));
#100038=CARTESIAN_POINT('Ctrl Pts',(18.2672434705536,21.2759258286182,-1.45875214605874));
#100039=CARTESIAN_POINT('Ctrl Pts',(18.2579262484274,21.2737976447271,-1.45818536554872));
#100040=CARTESIAN_POINT('Ctrl Pts',(18.2261829610988,21.2663205053888,-1.45625813426443));
#100041=CARTESIAN_POINT('Ctrl Pts',(18.2038295148217,21.260668227527,-1.4549074326959));
#100042=CARTESIAN_POINT('Ctrl Pts',(18.013001897462,21.2090848392155,-1.4434214562749));
#100043=CARTESIAN_POINT('Ctrl Pts',(17.8507182639555,21.1428388653696,-1.43402845751925));
#100044=CARTESIAN_POINT('Ctrl Pts',(17.6219897839229,21.0145513908651,-1.41976116469091));
#100045=CARTESIAN_POINT('Ctrl Pts',(17.5483186694448,20.9669959259469,-1.41496681028824));
#100046=CARTESIAN_POINT('Ctrl Pts',(17.4472435950924,20.8924842096476,-1.40779849604375));
#100047=CARTESIAN_POINT('Ctrl Pts',(17.4172897299615,20.8691329421779,-1.40559281767691));
#100048=CARTESIAN_POINT('Ctrl Pts',(17.3821311849691,20.8401707006092,-1.40288268092858));
#100049=CARTESIAN_POINT('Ctrl Pts',(17.3763062231969,20.8353195711646,-1.40242955688775));
#100050=CARTESIAN_POINT('Ctrl Pts',(17.36730672404,20.827742402918,-1.4017228434973));
#100051=CARTESIAN_POINT('Ctrl Pts',(17.3641139352504,20.8250380035354,-1.40147081003788));
#100052=CARTESIAN_POINT('Ctrl Pts',(17.3582169959043,20.8200129966435,-1.40100283890841));
#100053=CARTESIAN_POINT('Ctrl Pts',(17.3555106790074,20.81769502055,-1.40078709390854));
#100054=CARTESIAN_POINT('Ctrl Pts',(17.3494172701478,20.8124492525169,-1.40029912943574));
#100055=CARTESIAN_POINT('Ctrl Pts',(17.3460336263186,20.8095175597626,-1.40002662392805));
#100056=CARTESIAN_POINT('Ctrl Pts',(17.336107282698,20.8008617937674,-1.39922271670995));
#100057=CARTESIAN_POINT('Ctrl Pts',(17.3295906043254,20.795108208351,-1.39868919349516));
#100058=CARTESIAN_POINT('Ctrl Pts',(17.2837281587452,20.7541107583246,-1.39489464216436));
#100059=CARTESIAN_POINT('Ctrl Pts',(17.2456814511811,20.7174481782097,-1.39153841103967));
#100060=CARTESIAN_POINT('Ctrl Pts',(17.195507708285,20.6653423239044,-1.38686501604838));
#100061=CARTESIAN_POINT('Ctrl Pts',(17.1821618851296,20.6510932466922,-1.38559625206619));
#100062=CARTESIAN_POINT('Ctrl Pts',(17.0704045124053,20.5284143929947,-1.37476374100887));
#100063=CARTESIAN_POINT('Ctrl Pts',(16.9832811391905,20.4102161226442,-1.36495842821981));
#100064=CARTESIAN_POINT('Ctrl Pts',(16.8777709031625,20.2307611200807,-1.35150931276999));
#100065=CARTESIAN_POINT('Ctrl Pts',(16.8488256597699,20.1762036238822,-1.34758320436482));
#100066=CARTESIAN_POINT('Ctrl Pts',(16.8063135111892,20.0868420597404,-1.34141720810371));
#100067=CARTESIAN_POINT('Ctrl Pts',(16.7912114292737,20.0528119494022,-1.33912754783615));
#100068=CARTESIAN_POINT('Ctrl Pts',(16.7727688570564,20.0081105854558,-1.33619297680954));
#100069=CARTESIAN_POINT('Ctrl Pts',(16.7686050697038,19.9977881906051,-1.33552028771204));
#100070=CARTESIAN_POINT('Ctrl Pts',(16.7619671077403,19.9809505370373,-1.33443092601528));
#100071=CARTESIAN_POINT('Ctrl Pts',(16.759443395003,19.9744551546148,-1.33401258917509));
#100072=CARTESIAN_POINT('Ctrl Pts',(16.7546526297504,19.961942297938,-1.33321030082237));
#100073=CARTESIAN_POINT('Ctrl Pts',(16.752380836047,19.9559267329135,-1.33282619370624));
#100074=CARTESIAN_POINT('Ctrl Pts',(16.747243154446,19.9421326507232,-1.33194900818436));
#100075=CARTESIAN_POINT('Ctrl Pts',(16.7443954637851,19.9343474329577,-1.33145654214473));
#100076=CARTESIAN_POINT('Ctrl Pts',(16.7369541495323,19.9136274082932,-1.33015265068161));
#100077=CARTESIAN_POINT('Ctrl Pts',(16.7324404233318,19.9006641777291,-1.32934387929097));
#100078=CARTESIAN_POINT('Ctrl Pts',(16.6991412224389,19.8019489358526,-1.32323611985894));
#100079=CARTESIAN_POINT('Ctrl Pts',(16.6757502469573,19.7144696845719,-1.31812043168403));
#100080=CARTESIAN_POINT('Ctrl Pts',(16.6306361030139,19.4886587757842,-1.30537418782824));
#100081=CARTESIAN_POINT('Ctrl Pts',(16.6168948152935,19.3491947907301,-1.29793912363815));
#100082=CARTESIAN_POINT('Ctrl Pts',(16.6170159594101,19.1891094974785,-1.28909419861748));
#100083=CARTESIAN_POINT('Ctrl Pts',(16.6173229666296,19.1688226796989,-1.28796711911386));
#100084=CARTESIAN_POINT('Ctrl Pts',(16.6196735815231,19.0891814573856,-1.28350785079882));
#100085=CARTESIAN_POINT('Ctrl Pts',(16.6239226730702,19.0299246715509,-1.28011460872607));
#100086=CARTESIAN_POINT('Ctrl Pts',(16.6316702819436,18.9620446814946,-1.27606206003484));
#100087=CARTESIAN_POINT('Ctrl Pts',(16.6327408137148,18.9531651309176,-1.27552865258903));
#100088=CARTESIAN_POINT('Ctrl Pts',(16.6344383637347,18.9397981127848,-1.27472036792846));
#100089=CARTESIAN_POINT('Ctrl Pts',(16.6350235911771,18.9353053093828,-1.27444778944549));
#100090=CARTESIAN_POINT('Ctrl Pts',(16.636095341648,18.9272787126149,-1.27395914218773));
#100091=CARTESIAN_POINT('Ctrl Pts',(16.6365763775095,18.9237442393861,-1.27374338568322));
#100092=CARTESIAN_POINT('Ctrl Pts',(16.6376355523321,18.9161063336661,-1.27327586689139));
#100093=CARTESIAN_POINT('Ctrl Pts',(16.638216799053,18.9120034350728,-1.27302393636176));
#100094=CARTESIAN_POINT('Ctrl Pts',(16.6398690473806,18.9005821205774,-1.27232048023154));
#100095=CARTESIAN_POINT('Ctrl Pts',(16.6409663501364,18.8932676544505,-1.27186750771633));
#100096=CARTESIAN_POINT('Ctrl Pts',(16.6474610385354,18.8514691275068,-1.26926548143208));
#100097=CARTESIAN_POINT('Ctrl Pts',(16.6536719490448,18.8171191060285,-1.26707452535843));
#100098=CARTESIAN_POINT('Ctrl Pts',(16.6761041769704,18.708470376669,-1.26000955659443));
#100099=CARTESIAN_POINT('Ctrl Pts',(16.6954799621017,18.6348874107122,-1.25502391933505));
#100100=CARTESIAN_POINT('Ctrl Pts',(16.727155209449,18.5364540006172,-1.24820176212286));
#100101=CARTESIAN_POINT('Ctrl Pts',(16.736040526688,18.5105753721975,-1.24639313657688));
#100102=CARTESIAN_POINT('Ctrl Pts',(16.7454193884829,18.4848897112021,-1.2445862186816));
#100103=CARTESIAN_POINT('Origin',(18.734,19.211,0.));
#100104=CARTESIAN_POINT('',(16.7454194503191,18.4848895418526,-0.444429617362593));
#100105=CARTESIAN_POINT('',(16.7454194503191,18.4848895418526,-0.666446447912836));
#100106=CARTESIAN_POINT('',(16.7454194503191,18.4848895418526,0.));
#100107=CARTESIAN_POINT('',(20.3539256943887,20.5739122292573,0.));
#100108=CARTESIAN_POINT('Ctrl Pts',(16.7454194503191,18.4848895418526,-0.444429617362593));
#100109=CARTESIAN_POINT('Ctrl Pts',(16.770110946048,18.4172675601033,-0.440115253498862));
#100110=CARTESIAN_POINT('Ctrl Pts',(16.7982601300934,18.3508945674066,-0.435800889635131));
#100111=CARTESIAN_POINT('Ctrl Pts',(16.8297062688822,18.2861462896083,-0.4314865257714));
#100112=CARTESIAN_POINT('Ctrl Pts',(16.8611790966169,18.2213430586946,-0.427168500223636));
#100113=CARTESIAN_POINT('Ctrl Pts',(16.8959542522259,18.1581677454748,-0.422850474675871));
#100114=CARTESIAN_POINT('Ctrl Pts',(16.9338242035691,18.0969730245885,-0.418532449128106));
#100115=CARTESIAN_POINT('Ctrl Pts',(16.9717096236813,18.0357533074462,-0.414212659793034));
#100116=CARTESIAN_POINT('Ctrl Pts',(17.0126920735942,17.97651620248,-0.409892870457962));
#100117=CARTESIAN_POINT('Ctrl Pts',(17.0565212763453,17.9195844465527,-0.405573081122889));
#100118=CARTESIAN_POINT('Ctrl Pts',(17.100427251889,17.8625529669338,-0.401245725090954));
#100119=CARTESIAN_POINT('Ctrl Pts',(17.1471896162535,17.8078352797611,-0.396918369059018));
#100120=CARTESIAN_POINT('Ctrl Pts',(17.1965189481903,17.755719609379,-0.392591013027083));
#100121=CARTESIAN_POINT('Ctrl Pts',(17.2385584481092,17.71130553291,-0.38890314869949));
#100122=CARTESIAN_POINT('Ctrl Pts',(17.2824615181269,17.6687807432721,-0.385215284371896));
#100123=CARTESIAN_POINT('Ctrl Pts',(17.3280304443276,17.6283002152896,-0.381527420044303));
#100124=CARTESIAN_POINT('Ctrl Pts',(17.3823195172276,17.5800732650869,-0.37713383976892));
#100125=CARTESIAN_POINT('Ctrl Pts',(17.4391958858,17.5345513015008,-0.372740259493537));
#100126=CARTESIAN_POINT('Ctrl Pts',(17.4983592346194,17.4920232988986,-0.368346679218154));
#100127=CARTESIAN_POINT('Ctrl Pts',(17.5574362854365,17.4495573293242,-0.363959507592861));
#100128=CARTESIAN_POINT('Ctrl Pts',(17.6187933062776,17.4100769290324,-0.359572335967568));
#100129=CARTESIAN_POINT('Ctrl Pts',(17.6820956267706,17.3738320192261,-0.355185164342275));
#100130=CARTESIAN_POINT('Ctrl Pts',(17.7453254808102,17.3376286014228,-0.350803015009466));
#100131=CARTESIAN_POINT('Ctrl Pts',(17.810495795117,17.304653553715,-0.346420865676658));
#100132=CARTESIAN_POINT('Ctrl Pts',(17.8772429189521,17.2751135611627,-0.342038716343849));
#100133=CARTESIAN_POINT('Ctrl Pts',(17.9439489018955,17.245591776161,-0.337659268034262));
#100134=CARTESIAN_POINT('Ctrl Pts',(18.0122293270667,17.2195010391258,-0.333279819724674));
#100135=CARTESIAN_POINT('Ctrl Pts',(18.0816971982504,17.1970014759614,-0.328900371415087));
#100136=CARTESIAN_POINT('Ctrl Pts',(18.151144994395,17.1745084147899,-0.324522188691946));
#100137=CARTESIAN_POINT('Ctrl Pts',(18.2217790979678,17.155604615017,-0.320144005968804));
#100138=CARTESIAN_POINT('Ctrl Pts',(18.2931954157569,17.1404009759226,-0.315765823245663));
#100139=CARTESIAN_POINT('Ctrl Pts',(18.3646144753839,17.1251967531253,-0.311387472433939));
#100140=CARTESIAN_POINT('Ctrl Pts',(18.4368153380914,17.113693071257,-0.307009121622215));
#100141=CARTESIAN_POINT('Ctrl Pts',(18.5093833633923,17.1059497947652,-0.302630770810491));
#100142=CARTESIAN_POINT('Ctrl Pts',(18.5820273386455,17.0981984141328,-0.298247837601301));
#100143=CARTESIAN_POINT('Ctrl Pts',(18.6550387645182,17.09421534768,-0.293864904392111));
#100144=CARTESIAN_POINT('Ctrl Pts',(18.7279983301931,17.0940085073483,-0.289481971182921));
#100145=CARTESIAN_POINT('Ctrl Pts',(18.8009982495663,17.093801552614,-0.285096613787639));
#100146=CARTESIAN_POINT('Ctrl Pts',(18.8739457709894,17.0973749591399,-0.280711256392357));
#100147=CARTESIAN_POINT('Ctrl Pts',(18.9464247464519,17.1046845613501,-0.276325898997075));
#100148=CARTESIAN_POINT('Ctrl Pts',(19.0190318084556,17.1120070812603,-0.271932791695599));
#100149=CARTESIAN_POINT('Ctrl Pts',(19.0911681952094,17.1230789093043,-0.267539684394123));
#100150=CARTESIAN_POINT('Ctrl Pts',(19.1624265854903,17.1378044807966,-0.263146577092647));
#100151=CARTESIAN_POINT('Ctrl Pts',(19.209979484077,17.1476313040667,-0.260214922516055));
#100152=CARTESIAN_POINT('Ctrl Pts',(19.2571416240954,17.1590841897826,-0.257283267939462));
#100153=CARTESIAN_POINT('Ctrl Pts',(19.3037962299318,17.1721225499419,-0.254351613362869));
#100154=CARTESIAN_POINT('Ctrl Pts',(19.3728933426701,17.1914328200792,-0.250009729787665));
#100155=CARTESIAN_POINT('Ctrl Pts',(19.441158849408,17.2143020129624,-0.245667846212462));
#100156=CARTESIAN_POINT('Ctrl Pts',(19.5081940657064,17.2406415177372,-0.241325962637258));
#100157=CARTESIAN_POINT('Ctrl Pts',(19.575128336692,17.2669413590381,-0.236990617308954));
#100158=CARTESIAN_POINT('Ctrl Pts',(19.6408355376982,17.2967009666761,-0.232655271980649));
#100159=CARTESIAN_POINT('Ctrl Pts',(19.7049304637962,17.3297815027296,-0.228319926652345));
#100160=CARTESIAN_POINT('Ctrl Pts',(19.7689517228447,17.3628240179031,-0.223989564122503));
#100161=CARTESIAN_POINT('Ctrl Pts',(19.8313639491299,17.3991796603212,-0.219659201592662));
#100162=CARTESIAN_POINT('Ctrl Pts',(19.8918020078126,17.4386615699294,-0.21532883906282));
#100163=CARTESIAN_POINT('Ctrl Pts',(19.9522029223966,17.4781192146956,-0.211001137892668));
#100164=CARTESIAN_POINT('Ctrl Pts',(20.0106316627094,17.5206990484192,-0.206673436722516));
#100165=CARTESIAN_POINT('Ctrl Pts',(20.0667492121328,17.5661691462161,-0.202345735552364));
#100166=CARTESIAN_POINT('Ctrl Pts',(20.1228517146943,17.6116270520643,-0.198019194773624));
#100167=CARTESIAN_POINT('Ctrl Pts',(20.1766438725233,17.6599733741804,-0.193692653994883));
#100168=CARTESIAN_POINT('Ctrl Pts',(20.2278185824314,17.710934987148,-0.189366113216143));
#100169=CARTESIAN_POINT('Ctrl Pts',(20.2789973003963,17.7619005914824,-0.185039233578198));
#100170=CARTESIAN_POINT('Ctrl Pts',(20.3275578154845,17.8154815434691,-0.180712353940253));
#100171=CARTESIAN_POINT('Ctrl Pts',(20.3732301490776,17.8713681407361,-0.176385474302308));
#100172=CARTESIAN_POINT('Ctrl Pts',(20.4189572946786,17.9273218082918,-0.172053401915454));
#100173=CARTESIAN_POINT('Ctrl Pts',(20.4617890269818,17.9855862615223,-0.167721329528601));
#100174=CARTESIAN_POINT('Ctrl Pts',(20.5014965046459,18.0458197109183,-0.163389257141747));
#100175=CARTESIAN_POINT('Ctrl Pts',(20.5412284893311,18.1060903357408,-0.159054511047183));
#100176=CARTESIAN_POINT('Ctrl Pts',(20.5778321351825,18.1683319477764,-0.154719764952619));
#100177=CARTESIAN_POINT('Ctrl Pts',(20.6111242325247,18.2321774340216,-0.150385018858055));
#100178=CARTESIAN_POINT('Ctrl Pts',(20.6444833803135,18.2961515053878,-0.146041542563685));
#100179=CARTESIAN_POINT('Ctrl Pts',(20.6745174591996,18.3617354510943,-0.141698066269316));
#100180=CARTESIAN_POINT('Ctrl Pts',(20.7010913635959,18.4285419709235,-0.137354589974947));
#100181=CARTESIAN_POINT('Ctrl Pts',(20.7218496990689,18.480728210842,-0.133961662210443));
#100182=CARTESIAN_POINT('Ctrl Pts',(20.7404975995388,18.5336600360754,-0.130568734445939));
#100183=CARTESIAN_POINT('Ctrl Pts',(20.7569922795081,18.5871480648016,-0.127175806681435));
#100184=CARTESIAN_POINT('Ctrl Pts',(20.7789195363731,18.6582525510522,-0.12266540704014));
#100185=CARTESIAN_POINT('Ctrl Pts',(20.7971288498248,18.7306277670711,-0.118155007398845));
#100186=CARTESIAN_POINT('Ctrl Pts',(20.8114809457081,18.8038613010046,-0.113644607757551));
#100187=CARTESIAN_POINT('Ctrl Pts',(20.8265483310552,18.8807446973446,-0.108909415767653));
#100188=CARTESIAN_POINT('Ctrl Pts',(20.8373637791173,18.9585737514705,-0.104174223777755));
#100189=CARTESIAN_POINT('Ctrl Pts',(20.8438249692462,19.0368517897157,-0.0994390317878569));
#100190=CARTESIAN_POINT('Ctrl Pts',(20.8499589678183,19.1111658657987,-0.0949436276401115));
#100191=CARTESIAN_POINT('Ctrl Pts',(20.8521688918293,19.1858840436361,-0.0904482234923663));
#100192=CARTESIAN_POINT('Ctrl Pts',(20.8504195410052,19.2605714277716,-0.0859528193446209));
#100193=CARTESIAN_POINT('Ctrl Pts',(20.8486718350827,19.3351885839162,-0.0814616421919066));
#100194=CARTESIAN_POINT('Ctrl Pts',(20.8429722647592,19.4097745558195,-0.0769704650391922));
#100195=CARTESIAN_POINT('Ctrl Pts',(20.8333376405566,19.4838927828696,-0.0724792878864778));
#100196=CARTESIAN_POINT('Ctrl Pts',(20.8237095586262,19.5579606808563,-0.0679911604119481));
#100197=CARTESIAN_POINT('Ctrl Pts',(20.8101517936905,19.6315610202815,-0.0635030329374184));
#100198=CARTESIAN_POINT('Ctrl Pts',(20.7927330149949,19.7042619719479,-0.0590149054628886));
#100199=CARTESIAN_POINT('Ctrl Pts',(20.7753215178591,19.7769325324869,-0.0545286541571083));
#100200=CARTESIAN_POINT('Ctrl Pts',(20.7540523227982,19.8487040161605,-0.0500424028513279));
#100201=CARTESIAN_POINT('Ctrl Pts',(20.7290450048267,19.919155652887,-0.0455561515455476));
#100202=CARTESIAN_POINT('Ctrl Pts',(20.704034580516,19.9896160409194,-0.0410693429701386));
#100203=CARTESIAN_POINT('Ctrl Pts',(20.6752852491506,20.0587558278079,-0.0365825343947297));
#100204=CARTESIAN_POINT('Ctrl Pts',(20.642965902348,20.1261711226173,-0.0320957258193207));
#100205=CARTESIAN_POINT('Ctrl Pts',(20.6106450021441,20.1935896576844,-0.0276087015893536));
#100206=CARTESIAN_POINT('Ctrl Pts',(20.5747539463686,20.2592831330904,-0.0231216773593865));
#100207=CARTESIAN_POINT('Ctrl Pts',(20.5355083127276,20.3228708554384,-0.0186346531294194));
#100208=CARTESIAN_POINT('Ctrl Pts',(20.4962355967949,20.3865024578589,-0.0141445325320924));
#100209=CARTESIAN_POINT('Ctrl Pts',(20.4536039241545,20.448025026832,-0.00965441193476544));
#100210=CARTESIAN_POINT('Ctrl Pts',(20.4078726283013,20.5070861947508,-0.00516429133743847));
#100211=CARTESIAN_POINT('Ctrl Pts',(20.390340082504,20.5297291706837,-0.00344286089162564));
#100212=CARTESIAN_POINT('Ctrl Pts',(20.3723523809939,20.5520106992443,-0.00172143044581282));
#100213=CARTESIAN_POINT('Ctrl Pts',(20.3539256943887,20.5739122292573,0.));
#100214=CARTESIAN_POINT('',(17.1140596925741,20.5738948603531,-2.19263332840784E-7));
#100215=CARTESIAN_POINT('Origin',(18.734,19.211,0.));
#100216=CARTESIAN_POINT('Ctrl Pts',(17.1140596925741,20.5738948603531,-2.19263332840784E-7));
#100217=CARTESIAN_POINT('Ctrl Pts',(17.1607064305025,20.6293392920392,-0.00438522669745406));
#100218=CARTESIAN_POINT('Ctrl Pts',(17.2102945911145,20.6824950671961,-0.00877023413157529));
#100219=CARTESIAN_POINT('Ctrl Pts',(17.2625707969828,20.7330332126823,-0.0131552415656965));
#100220=CARTESIAN_POINT('Ctrl Pts',(17.3147693813981,20.7834963174456,-0.0175337379946171));
#100221=CARTESIAN_POINT('Ctrl Pts',(17.3696477435682,20.8313491749508,-0.0219122344235377));
#100222=CARTESIAN_POINT('Ctrl Pts',(17.4269127458042,20.8762963429729,-0.0262907308524583));
#100223=CARTESIAN_POINT('Ctrl Pts',(17.4841103523031,20.9211906122365,-0.0306640741864182));
#100224=CARTESIAN_POINT('Ctrl Pts',(17.5436886409257,20.9631856884276,-0.035037417520378));
#100225=CARTESIAN_POINT('Ctrl Pts',(17.6053194410708,21.0020246218004,-0.0394107608543379));
#100226=CARTESIAN_POINT('Ctrl Pts',(17.6669112432927,21.0408389791861,-0.0437813368818933));
#100227=CARTESIAN_POINT('Ctrl Pts',(17.7305525723989,21.0765008992431,-0.0481519129094486));
#100228=CARTESIAN_POINT('Ctrl Pts',(17.7958853222653,21.1087960510599,-0.052522488937004));
#100229=CARTESIAN_POINT('Ctrl Pts',(17.8611983685244,21.1410814630298,-0.0568917468490167));
#100230=CARTESIAN_POINT('Ctrl Pts',(17.9282013899052,21.1700019086928,-0.0612610047610293));
#100231=CARTESIAN_POINT('Ctrl Pts',(17.9965121600447,21.1953892475817,-0.065630262673042));
#100232=CARTESIAN_POINT('Ctrl Pts',(18.0648249509204,21.2207773374667,-0.069999649834335));
#100233=CARTESIAN_POINT('Ctrl Pts',(18.1344451137109,21.242631946831,-0.074369036995628));
#100234=CARTESIAN_POINT('Ctrl Pts',(18.2049725448516,21.260833883928,-0.078738424156921));
#100235=CARTESIAN_POINT('Ctrl Pts',(18.275571771191,21.2790543501514,-0.0831122592473974));
#100236=CARTESIAN_POINT('Ctrl Pts',(18.3470796408085,21.2936146004556,-0.0874860943378738));
#100237=CARTESIAN_POINT('Ctrl Pts',(18.4190839151667,21.3044461682865,-0.0918599294283503));
#100238=CARTESIAN_POINT('Ctrl Pts',(18.4911280120912,21.3152837266066,-0.0962361835049201));
#100239=CARTESIAN_POINT('Ctrl Pts',(18.5636685792402,21.322388450086,-0.10061243758149));
#100240=CARTESIAN_POINT('Ctrl Pts',(18.6362889712809,21.3257438508875,-0.10498869165806));
#100241=CARTESIAN_POINT('Ctrl Pts',(18.7090335036842,21.3291049875528,-0.109372426688018));
#100242=CARTESIAN_POINT('Ctrl Pts',(18.7818576501798,21.3287040083353,-0.113756161717976));
#100243=CARTESIAN_POINT('Ctrl Pts',(18.8543461708051,21.3245765420662,-0.118139896747934));
#100244=CARTESIAN_POINT('Ctrl Pts',(18.8963545400865,21.3221846029601,-0.120680348096389));
#100245=CARTESIAN_POINT('Ctrl Pts',(18.9382502971219,21.318542128427,-0.123220799444843));
#100246=CARTESIAN_POINT('Ctrl Pts',(18.9799541345816,21.3136639207639,-0.125761250793297));
#100247=CARTESIAN_POINT('Ctrl Pts',(19.0521147654861,21.3052231017867,-0.130157023059195));
#100248=CARTESIAN_POINT('Ctrl Pts',(19.1239757191856,21.2930474831033,-0.134552795325092));
#100249=CARTESIAN_POINT('Ctrl Pts',(19.1951211491521,21.2771694717047,-0.13894856759099));
#100250=CARTESIAN_POINT('Ctrl Pts',(19.2661637519632,21.2613144089446,-0.143337986606115));
#100251=CARTESIAN_POINT('Ctrl Pts',(19.336492418998,21.2417676813877,-0.14772740562124));
#100252=CARTESIAN_POINT('Ctrl Pts',(19.4056976665711,21.2186133205184,-0.152116824636366));
#100253=CARTESIAN_POINT('Ctrl Pts',(19.4748248958988,21.1954850626206,-0.156501295258381));
#100254=CARTESIAN_POINT('Ctrl Pts',(19.5428307683091,21.1687574028734,-0.160885765880396));
#100255=CARTESIAN_POINT('Ctrl Pts',(19.60931884804,21.1385647626645,-0.165270236502412));
#100256=CARTESIAN_POINT('Ctrl Pts',(19.6757666435217,21.1083904157775,-0.169652050631601));
#100257=CARTESIAN_POINT('Ctrl Pts',(19.7406980347465,21.0747554526423,-0.17403386476079));
#100258=CARTESIAN_POINT('Ctrl Pts',(19.8037358627713,21.0378426817602,-0.178415678889979));
#100259=CARTESIAN_POINT('Ctrl Pts',(19.8667560838771,21.0009402208808,-0.182796269146949));
#100260=CARTESIAN_POINT('Ctrl Pts',(19.9278833775877,20.9607620127547,-0.18717685940392));
#100261=CARTESIAN_POINT('Ctrl Pts',(19.9867660017252,20.9175363590974,-0.19155744966089));
#100262=CARTESIAN_POINT('Ctrl Pts',(20.0456514086938,20.8743086625677,-0.1959382469474));
#100263=CARTESIAN_POINT('Ctrl Pts',(20.1022915493499,20.828033520426,-0.20031904423391));
#100264=CARTESIAN_POINT('Ctrl Pts',(20.1563657971912,20.7789810391011,-0.20469984152042));
#100265=CARTESIAN_POINT('Ctrl Pts',(20.2104971638002,20.7298767435135,-0.209085266254415));
#100266=CARTESIAN_POINT('Ctrl Pts',(20.2620568697778,20.6779895750516,-0.213470690988409));
#100267=CARTESIAN_POINT('Ctrl Pts',(20.3107599897288,20.6236276702623,-0.217856115722404));
#100268=CARTESIAN_POINT('Ctrl Pts',(20.3594903544991,20.569235355095,-0.222243993689482));
#100269=CARTESIAN_POINT('Ctrl Pts',(20.4053606496669,20.5123659213336,-0.226631871656561));
#100270=CARTESIAN_POINT('Ctrl Pts',(20.4481269507232,20.4533597694728,-0.23101974962364));
#100271=CARTESIAN_POINT('Ctrl Pts',(20.4909689880789,20.3942491216075,-0.235415398233292));
#100272=CARTESIAN_POINT('Ctrl Pts',(20.5306957923997,20.3329946025317,-0.239811046842944));
#100273=CARTESIAN_POINT('Ctrl Pts',(20.5671076961722,20.2699641987499,-0.244206695452596));
#100274=CARTESIAN_POINT('Ctrl Pts',(20.5912140439174,20.2282351850303,-0.247116816126641));
#100275=CARTESIAN_POINT('Ctrl Pts',(20.613868403521,20.1857283140019,-0.250026936800686));
#100276=CARTESIAN_POINT('Ctrl Pts',(20.6350244604073,20.1425551518472,-0.252937057474731));
#100277=CARTESIAN_POINT('Ctrl Pts',(20.6668851126084,20.0775371236191,-0.257319648387443));
#100278=CARTESIAN_POINT('Ctrl Pts',(20.6954700480251,20.010752620059,-0.261702239300154));
#100279=CARTESIAN_POINT('Ctrl Pts',(20.720580205096,19.9425655054202,-0.266084830212866));
#100280=CARTESIAN_POINT('Ctrl Pts',(20.745652583015,19.8744809807951,-0.270460827356882));
#100281=CARTESIAN_POINT('Ctrl Pts',(20.7672603940222,19.8049984839898,-0.274836824500899));
#100282=CARTESIAN_POINT('Ctrl Pts',(20.7852512551748,19.7345048119585,-0.279212821644915));
#100283=CARTESIAN_POINT('Ctrl Pts',(20.8032205628375,19.6640955930635,-0.283583576237753));
#100284=CARTESIAN_POINT('Ctrl Pts',(20.8175814089924,19.5926780716228,-0.287954330830591));
#100285=CARTESIAN_POINT('Ctrl Pts',(20.8282307375361,19.520655644158,-0.292325085423429));
#100286=CARTESIAN_POINT('Ctrl Pts',(20.8388731698584,19.4486798564986,-0.296693009632021));
#100287=CARTESIAN_POINT('Ctrl Pts',(20.845808782324,19.3761004173276,-0.301060933840613));
#100288=CARTESIAN_POINT('Ctrl Pts',(20.8489855761766,19.3033309946066,-0.305428858049204));
#100289=CARTESIAN_POINT('Ctrl Pts',(20.8521613682029,19.2305845202815,-0.309795404799378));
#100290=CARTESIAN_POINT('Ctrl Pts',(20.8515806736046,19.157648664371,-0.314161951549551));
#100291=CARTESIAN_POINT('Ctrl Pts',(20.8472434850165,19.0849405971962,-0.318528498299725));
#100292=CARTESIAN_POINT('Ctrl Pts',(20.842906223341,19.0122313047932,-0.32289511863205));
#100293=CARTESIAN_POINT('Ctrl Pts',(20.8348123728149,18.939750291573,-0.327261738964374));
#100294=CARTESIAN_POINT('Ctrl Pts',(20.8230139324319,18.8679113961303,-0.331628359296699));
#100295=CARTESIAN_POINT('Ctrl Pts',(20.8112032798744,18.7959981426279,-0.335999499373007));
#100296=CARTESIAN_POINT('Ctrl Pts',(20.7956804601328,18.7247288123433,-0.340370639449314));
#100297=CARTESIAN_POINT('Ctrl Pts',(20.7765488036571,18.654507965305,-0.344741779525621));
#100298=CARTESIAN_POINT('Ctrl Pts',(20.7574067702789,18.5842490308754,-0.349115290483651));
#100299=CARTESIAN_POINT('Ctrl Pts',(20.7346521545122,18.5150401717766,-0.353488801441681));
#100300=CARTESIAN_POINT('Ctrl Pts',(20.7084376488589,18.4472690455607,-0.35786231239971));
#100301=CARTESIAN_POINT('Ctrl Pts',(20.6821764073163,18.3793770952527,-0.362243620564609));
#100302=CARTESIAN_POINT('Ctrl Pts',(20.6524431558452,18.31292843841,-0.366624928729508));
#100303=CARTESIAN_POINT('Ctrl Pts',(20.6194377827199,18.2482885336238,-0.371006236894407));
#100304=CARTESIAN_POINT('Ctrl Pts',(20.5965703635706,18.2035034681465,-0.374041779314993));
#100305=CARTESIAN_POINT('Ctrl Pts',(20.572133215651,18.1595861430692,-0.37707732173558));
#100306=CARTESIAN_POINT('Ctrl Pts',(20.54620485702,18.1166497104705,-0.380112864156166));
#100307=CARTESIAN_POINT('Ctrl Pts',(20.5087129403854,18.0545644402657,-0.384502201136292));
#100308=CARTESIAN_POINT('Ctrl Pts',(20.4679538797132,17.9942872987423,-0.388891538116418));
#100309=CARTESIAN_POINT('Ctrl Pts',(20.4241274618398,17.9361830865827,-0.393280875096543));
#100310=CARTESIAN_POINT('Ctrl Pts',(20.3803660305827,17.8781650324146,-0.397663703487278));
#100311=CARTESIAN_POINT('Ctrl Pts',(20.3335465592593,17.8223138929918,-0.402046531878012));
#100312=CARTESIAN_POINT('Ctrl Pts',(20.2839133009206,17.7689674900928,-0.406429360268747));
#100313=CARTESIAN_POINT('Ctrl Pts',(20.2343383423802,17.7156837484943,-0.410807040538664));
#100314=CARTESIAN_POINT('Ctrl Pts',(20.1819564893205,17.6648992500388,-0.415184720808581));
#100315=CARTESIAN_POINT('Ctrl Pts',(20.127052568789,17.616919217671,-0.419562401078499));
#100316=CARTESIAN_POINT('Ctrl Pts',(20.0721834605648,17.5689696074592,-0.423937305642242));
#100317=CARTESIAN_POINT('Ctrl Pts',(20.0147958199512,17.5238212515477,-0.428312210205985));
#100318=CARTESIAN_POINT('Ctrl Pts',(19.9552106611291,17.4817419159811,-0.432687114769728));
#100319=CARTESIAN_POINT('Ctrl Pts',(19.8956436547536,17.4396753997626,-0.437060686531434));
#100320=CARTESIAN_POINT('Ctrl Pts',(19.8338808528525,17.4006763255856,-0.44143425829314));
#100321=CARTESIAN_POINT('Ctrl Pts',(19.7702742782371,17.3649705797945,-0.445807830054846));
#100322=CARTESIAN_POINT('Ctrl Pts',(19.706666129022,17.3292639500971,-0.450181510085624));
#100323=CARTESIAN_POINT('Ctrl Pts',(19.6412145378353,17.2968510448943,-0.454555190116402));
#100324=CARTESIAN_POINT('Ctrl Pts',(19.5742968108292,17.2679121816783,-0.45892887014718));
#100325=CARTESIAN_POINT('Ctrl Pts',(19.5073098565464,17.2389433808242,-0.463307074808002));
#100326=CARTESIAN_POINT('Ctrl Pts',(19.4388541815959,17.2134559893026,-0.467685279468823));
#100327=CARTESIAN_POINT('Ctrl Pts',(19.3693270226857,17.191582119955,-0.472063484129645));
#100328=CARTESIAN_POINT('Ctrl Pts',(19.2997619936054,17.1696963363115,-0.476444073518358));
#100329=CARTESIAN_POINT('Ctrl Pts',(19.2291247856183,17.1514281144628,-0.480824662907072));
#100330=CARTESIAN_POINT('Ctrl Pts',(19.1578251136208,17.1368589071463,-0.485205252295786));
#100331=CARTESIAN_POINT('Ctrl Pts',(19.0863994489354,17.1222639547802,-0.489593582564878));
#100332=CARTESIAN_POINT('Ctrl Pts',(19.0143094596386,17.1113811421464,-0.49398191283397));
#100333=CARTESIAN_POINT('Ctrl Pts',(18.9419717193455,17.1042402215838,-0.498370243103063));
#100334=CARTESIAN_POINT('Ctrl Pts',(18.8929675902332,17.0994027108761,-0.501343052347909));
#100335=CARTESIAN_POINT('Ctrl Pts',(18.8438498553954,17.0962813345305,-0.504315861592754));
#100336=CARTESIAN_POINT('Ctrl Pts',(18.7947475345845,17.0948717578932,-0.5072886708376));
#100337=CARTESIAN_POINT('Ctrl Pts',(18.7222522737112,17.0927906418817,-0.511677762395248));
#100338=CARTESIAN_POINT('Ctrl Pts',(18.6495091103977,17.0944351532161,-0.516066853952897));
#100339=CARTESIAN_POINT('Ctrl Pts',(18.5769329023863,17.0998346993077,-0.520455945510545));
#100340=CARTESIAN_POINT('Ctrl Pts',(18.5044640605617,17.1052262575382,-0.524838544030911));
#100341=CARTESIAN_POINT('Ctrl Pts',(18.4321621606072,17.1143617873598,-0.529221142551278));
#100342=CARTESIAN_POINT('Ctrl Pts',(18.3604434342997,17.1272187033611,-0.533603741071644));
#100343=CARTESIAN_POINT('Ctrl Pts',(18.2888085527943,17.1400605886216,-0.537981215991463));
#100344=CARTESIAN_POINT('Ctrl Pts',(18.2177559628244,17.1566151328626,-0.542358690911283));
#100345=CARTESIAN_POINT('Ctrl Pts',(18.1476964397083,17.1768079895965,-0.546736165831102));
#100346=CARTESIAN_POINT('Ctrl Pts',(18.0776810968814,17.1969881124977,-0.551110880268134));
#100347=CARTESIAN_POINT('Ctrl Pts',(18.0086580405141,17.2208018623067,-0.555485594705165));
#100348=CARTESIAN_POINT('Ctrl Pts',(17.9410261268036,17.2481241923066,-0.559860309142197));
#100349=CARTESIAN_POINT('Ctrl Pts',(17.8734145775147,17.2754382953703,-0.564233706323445));
#100350=CARTESIAN_POINT('Ctrl Pts',(17.8071937860416,17.3062587006989,-0.568607103504694));
#100351=CARTESIAN_POINT('Ctrl Pts',(17.742744167297,17.340411623544,-0.572980500685942));
#100352=CARTESIAN_POINT('Ctrl Pts',(17.6782927189291,17.3745655159369,-0.577354022021053));
#100353=CARTESIAN_POINT('Ctrl Pts',(17.6156129682129,17.4120518861517,-0.581727543356163));
#100354=CARTESIAN_POINT('Ctrl Pts',(17.5550606878344,17.4526510305885,-0.586101064691274));
#100355=CARTESIAN_POINT('Ctrl Pts',(17.4944454063011,17.4932924160932,-0.590479136423054));
#100356=CARTESIAN_POINT('Ctrl Pts',(17.435962415829,17.5370527729163,-0.594857208154835));
#100357=CARTESIAN_POINT('Ctrl Pts',(17.3799377355334,17.5836695529341,-0.599235279886616));
#100358=CARTESIAN_POINT('Ctrl Pts',(17.3238823567118,17.6303118764521,-0.603615750567369));
#100359=CARTESIAN_POINT('Ctrl Pts',(17.2702883244171,17.6798134120468,-0.607996221248123));
#100360=CARTESIAN_POINT('Ctrl Pts',(17.2194458037231,17.7318737083872,-0.612376691928877));
#100361=CARTESIAN_POINT('Ctrl Pts',(17.1685131538602,17.7840262926627,-0.616764927924507));
#100362=CARTESIAN_POINT('Ctrl Pts',(17.1203420749117,17.8387463335722,-0.621153163920137));
#100363=CARTESIAN_POINT('Ctrl Pts',(17.0751829640465,17.895699638398,-0.625541399915768));
#100364=CARTESIAN_POINT('Ctrl Pts',(17.0445739865328,17.9343027550967,-0.628515759116857));
#100365=CARTESIAN_POINT('Ctrl Pts',(17.0153478916349,17.9739312043245,-0.631490118317945));
#100366=CARTESIAN_POINT('Ctrl Pts',(16.9875709408017,18.0144739696991,-0.634464477519034));
#100367=CARTESIAN_POINT('Ctrl Pts',(16.946006537119,18.0751406669388,-0.638915198812158));
#100368=CARTESIAN_POINT('Ctrl Pts',(16.9075293793436,18.1380885815645,-0.643365920105282));
#100369=CARTESIAN_POINT('Ctrl Pts',(16.8723941622653,18.202975841107,-0.647816641398406));
#100370=CARTESIAN_POINT('Ctrl Pts',(16.8373240418129,18.2677428810517,-0.652259116636339));
#100371=CARTESIAN_POINT('Ctrl Pts',(16.8055837739661,18.3344417187871,-0.656701591874273));
#100372=CARTESIAN_POINT('Ctrl Pts',(16.7773849587093,18.4027014288056,-0.661144067112207));
#100373=CARTESIAN_POINT('Ctrl Pts',(16.7661659236286,18.4298588846888,-0.662911527379083));
#100374=CARTESIAN_POINT('Ctrl Pts',(16.7555069732342,18.4572630951622,-0.66467898764596));
#100375=CARTESIAN_POINT('Ctrl Pts',(16.7454194503191,18.4848895418526,-0.666446447912836));
#100376=CARTESIAN_POINT('Origin',(-18.734,19.211,0.));
#100377=CARTESIAN_POINT('',(-20.7225806138391,18.4848897175613,-21.2464098975766));
#100378=CARTESIAN_POINT('',(-20.7225806137704,18.4848897173731,-21.4658225507677));
#100379=CARTESIAN_POINT('',(-20.7225806137986,18.4848897174502,0.));
#100380=CARTESIAN_POINT('',(-20.8509993841528,19.2093852254739,-21.5109437210328));
#100381=CARTESIAN_POINT('Ctrl Pts',(-20.7225806137704,18.4848897173731,
-21.4658225507677));
#100382=CARTESIAN_POINT('Ctrl Pts',(-20.7235160649965,18.4874516149495,
-21.4659708387453));
#100383=CARTESIAN_POINT('Ctrl Pts',(-20.7244465747682,18.4900153457236,
-21.4661191633266));
#100384=CARTESIAN_POINT('Ctrl Pts',(-20.7392648735409,18.5310899038959,
-21.4684945105102));
#100385=CARTESIAN_POINT('Ctrl Pts',(-20.752037343799,18.5699929221988,-21.4707297776479));
#100386=CARTESIAN_POINT('Ctrl Pts',(-20.769047825713,18.6273675720992,-21.4740351573867));
#100387=CARTESIAN_POINT('Ctrl Pts',(-20.7741789047585,18.6455652346253,
-21.4750848285083));
#100388=CARTESIAN_POINT('Ctrl Pts',(-20.7946969717739,18.7222520054448,
-21.47952257391));
#100389=CARTESIAN_POINT('Ctrl Pts',(-20.8078162681752,18.7813126039396,
-21.4829748366309));
#100390=CARTESIAN_POINT('Ctrl Pts',(-20.8199723987728,18.849765732952,-21.4870988243204));
#100391=CARTESIAN_POINT('Ctrl Pts',(-20.821498852619,18.8586939146429,-21.4876390876925));
#100392=CARTESIAN_POINT('Ctrl Pts',(-20.8236942930998,18.8720504219912,
-21.4884512443157));
#100393=CARTESIAN_POINT('Ctrl Pts',(-20.8244066210205,18.8764716559285,
-21.4887207236647));
#100394=CARTESIAN_POINT('Ctrl Pts',(-20.8256595713244,18.8844086792473,
-21.4892056988168));
#100395=CARTESIAN_POINT('Ctrl Pts',(-20.8262053651736,18.887923596436,-21.4894208972808));
#100396=CARTESIAN_POINT('Ctrl Pts',(-20.8272520064275,18.8947778637196,
-21.4898413773222));
#100397=CARTESIAN_POINT('Ctrl Pts',(-20.8277537217311,18.8981170278596,
-21.4900466025942));
#100398=CARTESIAN_POINT('Ctrl Pts',(-20.8288494645378,18.905530405555,-21.4905030547554));
#100399=CARTESIAN_POINT('Ctrl Pts',(-20.8294395976159,18.9096051687625,
-21.4907544964867));
#100400=CARTESIAN_POINT('Ctrl Pts',(-20.8308794579733,18.9197558115371,
-21.4913821951212));
#100401=CARTESIAN_POINT('Ctrl Pts',(-20.8317146611703,18.9258336681553,
-21.4917592268512));
#100402=CARTESIAN_POINT('Ctrl Pts',(-20.8356021208692,18.9550646364502,
-21.4935779570296));
#100403=CARTESIAN_POINT('Ctrl Pts',(-20.8382974076893,18.9782625879247,
-21.4950376552817));
#100404=CARTESIAN_POINT('Ctrl Pts',(-20.8474812625982,19.0706096824942,
-21.5009009210641));
#100405=CARTESIAN_POINT('Ctrl Pts',(-20.8509485247462,19.1400100451708,
-21.505422601223));
#100406=CARTESIAN_POINT('Ctrl Pts',(-20.8509994310935,19.209447985236,-21.5099894778226));
#100407=CARTESIAN_POINT('',(-17.1140743056112,17.8480877707428,-22.));
#100408=CARTESIAN_POINT('Ctrl Pts',(-20.8509993841528,19.2093852254739,
-21.5109437210328));
#100409=CARTESIAN_POINT('Ctrl Pts',(-20.8510560152528,19.2836296489979,
-21.5154240901546));
#100410=CARTESIAN_POINT('Ctrl Pts',(-20.8472020809542,19.3580185555351,
-21.5199044592764));
#100411=CARTESIAN_POINT('Ctrl Pts',(-20.8394225376055,19.4320993852161,
-21.5243848283982));
#100412=CARTESIAN_POINT('Ctrl Pts',(-20.8319236730415,19.5035074465459,
-21.5287035499137));
#100413=CARTESIAN_POINT('Ctrl Pts',(-20.8207776605642,19.5746287335346,
-21.5330222714292));
#100414=CARTESIAN_POINT('Ctrl Pts',(-20.8060239446483,19.6450573381528,
-21.5373409929446));
#100415=CARTESIAN_POINT('Ctrl Pts',(-20.7912800573181,19.7154390248567,
-21.5416568374273));
#100416=CARTESIAN_POINT('Ctrl Pts',(-20.7729333327059,19.7851284592732,
-21.54597268191));
#100417=CARTESIAN_POINT('Ctrl Pts',(-20.751074714518,19.85372746639,-21.5502885263927));
#100418=CARTESIAN_POINT('Ctrl Pts',(-20.7292229871427,19.9223048480364,
-21.5546030103284));
#100419=CARTESIAN_POINT('Ctrl Pts',(-20.7038617135749,19.989792011532,-21.5589174942642));
#100420=CARTESIAN_POINT('Ctrl Pts',(-20.6751318580095,20.0558053680112,
-21.5632319782));
#100421=CARTESIAN_POINT('Ctrl Pts',(-20.6464009777761,20.1218210788973,
-21.5675466160145));
#100422=CARTESIAN_POINT('Ctrl Pts',(-20.6143014783329,20.1863624243994,
-21.5718612538289));
#100423=CARTESIAN_POINT('Ctrl Pts',(-20.5790219329057,20.2490669858429,
-21.5761758916434));
#100424=CARTESIAN_POINT('Ctrl Pts',(-20.5437074985004,20.3118335576677,
-21.5804947963299));
#100425=CARTESIAN_POINT('Ctrl Pts',(-20.5052069895562,20.3727592890194,
-21.5848137010164));
#100426=CARTESIAN_POINT('Ctrl Pts',(-20.4637537248945,20.4315085215654,
-21.5891326057028));
#100427=CARTESIAN_POINT('Ctrl Pts',(-20.4222758047099,20.490292696909,-21.5934540791822));
#100428=CARTESIAN_POINT('Ctrl Pts',(-20.3778419441492,20.5468974099959,
-21.5977755526616));
#100429=CARTESIAN_POINT('Ctrl Pts',(-20.3307256309594,20.6010202370604,
-21.602097026141));
#100430=CARTESIAN_POINT('Ctrl Pts',(-20.2835347289174,20.6552287448428,
-21.6064253408548));
#100431=CARTESIAN_POINT('Ctrl Pts',(-20.2336532518318,20.7069471772808,
-21.6107536555687));
#100432=CARTESIAN_POINT('Ctrl Pts',(-20.1813905512658,20.7559108686608,
-21.6150819702825));
#100433=CARTESIAN_POINT('Ctrl Pts',(-20.1677437911292,20.7686961963311,
-21.6162121735069));
#100434=CARTESIAN_POINT('Ctrl Pts',(-20.1539348377413,20.7812939190609,
-21.6173423767313));
#100435=CARTESIAN_POINT('Ctrl Pts',(-20.1399695343548,20.7936998036476,
-21.6184725799557));
#100436=CARTESIAN_POINT('Ctrl Pts',(-20.0856806209083,20.8419266108937,
-21.6228661475946));
#100437=CARTESIAN_POINT('Ctrl Pts',(-20.0288044225739,20.8874484514207,
-21.6272597152335));
#100438=CARTESIAN_POINT('Ctrl Pts',(-19.969641252187,20.9299763511735,-21.6316532828724));
#100439=CARTESIAN_POINT('Ctrl Pts',(-19.9105643807625,20.9724422171713,
-21.6360404417891));
#100440=CARTESIAN_POINT('Ctrl Pts',(-19.8492075475795,21.0119225341567,
-21.6404276007057));
#100441=CARTESIAN_POINT('Ctrl Pts',(-19.7859054205823,21.0481673810923,
-21.6448147596223));
#100442=CARTESIAN_POINT('Ctrl Pts',(-19.7226757606735,21.0843707356065,
-21.6491968962016));
#100443=CARTESIAN_POINT('Ctrl Pts',(-19.6575056463758,21.1173457404982,
-21.6535790327809));
#100444=CARTESIAN_POINT('Ctrl Pts',(-19.5907587261481,21.1468857107715,
-21.6579611693603));
#100445=CARTESIAN_POINT('Ctrl Pts',(-19.5240529471153,21.1764074733181,
-21.6623406048961));
#100446=CARTESIAN_POINT('Ctrl Pts',(-19.4557727294709,21.2024982084515,
-21.6667200404319));
#100447=CARTESIAN_POINT('Ctrl Pts',(-19.3863050672729,21.2249977902694,
-21.6710994759677));
#100448=CARTESIAN_POINT('Ctrl Pts',(-19.3168574801292,21.2474908700645,
-21.675477645916));
#100449=CARTESIAN_POINT('Ctrl Pts',(-19.2462235870207,21.2663947090105,
-21.6798558158643));
#100450=CARTESIAN_POINT('Ctrl Pts',(-19.1748074790919,21.2815984077982,
-21.6842339858126));
#100451=CARTESIAN_POINT('Ctrl Pts',(-19.1033886290296,21.2968026903559,
-21.6886123238676));
#100452=CARTESIAN_POINT('Ctrl Pts',(-19.0311879752792,21.3083064524741,
-21.6929906619226));
#100453=CARTESIAN_POINT('Ctrl Pts',(-18.9586201563122,21.3160498296663,
-21.6973689999776));
#100454=CARTESIAN_POINT('Ctrl Pts',(-18.8859763854436,21.3238013113356,
-21.7017519205474));
#100455=CARTESIAN_POINT('Ctrl Pts',(-18.8129651613081,21.3277844990936,
-21.7061348411171));
#100456=CARTESIAN_POINT('Ctrl Pts',(-18.740005792739,21.3279914809591,-21.7105177616869));
#100457=CARTESIAN_POINT('Ctrl Pts',(-18.667006069685,21.3281985773082,-21.7149031064896));
#100458=CARTESIAN_POINT('Ctrl Pts',(-18.594058739949,21.324625332556,-21.7192884512922));
#100459=CARTESIAN_POINT('Ctrl Pts',(-18.5215799495222,21.3173159122399,
-21.7236737960949));
#100460=CARTESIAN_POINT('Ctrl Pts',(-18.4489730689546,21.3099935741492,
-21.7280668910191));
#100461=CARTESIAN_POINT('Ctrl Pts',(-18.3768368570158,21.2989219477122,
-21.7324599859433));
#100462=CARTESIAN_POINT('Ctrl Pts',(-18.3055786328722,21.284196597573,-21.7368530808674));
#100463=CARTESIAN_POINT('Ctrl Pts',(-18.2580238618235,21.2743695121678,
-21.7397848494573));
#100464=CARTESIAN_POINT('Ctrl Pts',(-18.2108598781006,21.2629162374028,
-21.7427166180472));
#100465=CARTESIAN_POINT('Ctrl Pts',(-18.1642034712006,21.2498773665349,
-21.7456483866371));
#100466=CARTESIAN_POINT('Ctrl Pts',(-18.0951059728948,21.230566977725,-21.7499902956831));
#100467=CARTESIAN_POINT('Ctrl Pts',(-18.0268401014068,21.2076976293853,
-21.754332204729));
#100468=CARTESIAN_POINT('Ctrl Pts',(-17.959804544219,21.1813579360736,-21.758674113775));
#100469=CARTESIAN_POINT('Ctrl Pts',(-17.8928699309423,21.1550579057671,
-21.7630094846598));
#100470=CARTESIAN_POINT('Ctrl Pts',(-17.8271624114981,21.1252980759476,
-21.7673448555445));
#100471=CARTESIAN_POINT('Ctrl Pts',(-17.7630671934661,21.0922172881398,
-21.7716802264293));
#100472=CARTESIAN_POINT('Ctrl Pts',(-17.6990456418676,21.0591745210102,
-21.7760106145506));
#100473=CARTESIAN_POINT('Ctrl Pts',(-17.6366331495171,21.0228185970339,
-21.7803410026719));
#100474=CARTESIAN_POINT('Ctrl Pts',(-17.5761948535926,20.9833363797407,
-21.7846713907932));
#100475=CARTESIAN_POINT('Ctrl Pts',(-17.5157937013986,20.9438784271429,
-21.7889991175759));
#100476=CARTESIAN_POINT('Ctrl Pts',(-17.4573647522916,20.9012982594394,
-21.7933268443586));
#100477=CARTESIAN_POINT('Ctrl Pts',(-17.4012470250051,20.8558278048605,
-21.7976545711413));
#100478=CARTESIAN_POINT('Ctrl Pts',(-17.3451443445715,20.81036954228,-21.8019811375301));
#100479=CARTESIAN_POINT('Ctrl Pts',(-17.2913520397843,20.7620228406339,
-21.8063077039189));
#100480=CARTESIAN_POINT('Ctrl Pts',(-17.2401772158046,20.7110608285729,
-21.8106342703077));
#100481=CARTESIAN_POINT('Ctrl Pts',(-17.1889983840908,20.6600948254439,
-21.8149611755297));
#100482=CARTESIAN_POINT('Ctrl Pts',(-17.1404377881069,20.6065134551268,
-21.8192880807517));
#100483=CARTESIAN_POINT('Ctrl Pts',(-17.0947654083712,20.5506264231522,
-21.8236149859736));
#100484=CARTESIAN_POINT('Ctrl Pts',(-17.0490382189606,20.4946723232895,
-21.827947083749));
#100485=CARTESIAN_POINT('Ctrl Pts',(-17.0062064773784,20.4364074215726,
-21.8322791815243));
#100486=CARTESIAN_POINT('Ctrl Pts',(-16.9664990268283,20.3761735106142,
-21.8366112792996));
#100487=CARTESIAN_POINT('Ctrl Pts',(-16.9267670699395,20.3159024249543,
-21.8409460507257));
#100488=CARTESIAN_POINT('Ctrl Pts',(-16.8901634882159,20.2536603390498,
-21.8452808221518));
#100489=CARTESIAN_POINT('Ctrl Pts',(-16.856871493227,20.1898143690508,-21.8496155935779));
#100490=CARTESIAN_POINT('Ctrl Pts',(-16.8235124512874,20.1258398192654,
-21.8539590948264));
#100491=CARTESIAN_POINT('Ctrl Pts',(-16.7934785159735,20.060255385527,-21.858302596075));
#100492=CARTESIAN_POINT('Ctrl Pts',(-16.7669047947946,19.9934483712413,
-21.8626460973235));
#100493=CARTESIAN_POINT('Ctrl Pts',(-16.7461481233425,19.9412655686561,
-21.8660387959885));
#100494=CARTESIAN_POINT('Ctrl Pts',(-16.7275016016086,19.8883372861217,
-21.8694314946536));
#100495=CARTESIAN_POINT('Ctrl Pts',(-16.7110080073322,19.8348528653473,
-21.8728241933186));
#100496=CARTESIAN_POINT('Ctrl Pts',(-16.6890808041098,19.7637486691424,
-21.8773345742491));
#100497=CARTESIAN_POINT('Ctrl Pts',(-16.6708715122103,19.691373744136,-21.8818449551797));
#100498=CARTESIAN_POINT('Ctrl Pts',(-16.6565194069635,19.6181404985465,
-21.8863553361102));
#100499=CARTESIAN_POINT('Ctrl Pts',(-16.6414519418388,19.5412570480063,
-21.891090530439));
#100500=CARTESIAN_POINT('Ctrl Pts',(-16.6306364194547,19.4634279279486,
-21.8958257247677));
#100501=CARTESIAN_POINT('Ctrl Pts',(-16.6241751632239,19.3851498151671,
-21.9005609190965));
#100502=CARTESIAN_POINT('Ctrl Pts',(-16.618041130639,19.3108360165285,-21.9050563044009));
#100503=CARTESIAN_POINT('Ctrl Pts',(-16.6158311432077,19.2361181121913,
-21.9095516897054));
#100504=CARTESIAN_POINT('Ctrl Pts',(-16.6175804022592,19.1614309945752,
-21.9140470750099));
#100505=CARTESIAN_POINT('Ctrl Pts',(-16.6193280165078,19.0868141041766,
-21.9185382333685));
#100506=CARTESIAN_POINT('Ctrl Pts',(-16.6250274669155,19.0122283910569,
-21.9230293917272));
#100507=CARTESIAN_POINT('Ctrl Pts',(-16.6346619440205,18.9381104129575,
-21.9275205500858));
#100508=CARTESIAN_POINT('Ctrl Pts',(-16.644289879149,18.8640427622465,-21.9320086588702));
#100509=CARTESIAN_POINT('Ctrl Pts',(-16.6578474702978,18.7904426603016,
-21.9364967676547));
#100510=CARTESIAN_POINT('Ctrl Pts',(-16.6752660492705,18.7177419335545,
-21.9409848764392));
#100511=CARTESIAN_POINT('Ctrl Pts',(-16.6926773473537,18.6450715953915,
-21.9454711092139));
#100512=CARTESIAN_POINT('Ctrl Pts',(-16.7139463177063,18.5733003216091,
-21.9499573419886));
#100513=CARTESIAN_POINT('Ctrl Pts',(-16.7389533863518,18.5028488795668,
-21.9544435747634));
#100514=CARTESIAN_POINT('Ctrl Pts',(-16.7639635634828,18.432388680109,-21.958930365196));
#100515=CARTESIAN_POINT('Ctrl Pts',(-16.7927126236932,18.363249066819,-21.9634171556287));
#100516=CARTESIAN_POINT('Ctrl Pts',(-16.8250316763889,18.2958339279402,
-21.9679039460613));
#100517=CARTESIAN_POINT('Ctrl Pts',(-16.8573522841798,18.2284155452484,
-21.9723909523848));
#100518=CARTESIAN_POINT('Ctrl Pts',(-16.8932430249613,18.1627222047342,
-21.9768779587083));
#100519=CARTESIAN_POINT('Ctrl Pts',(-16.9324883220855,18.0991345970228,
-21.9813649650317));
#100520=CARTESIAN_POINT('Ctrl Pts',(-16.9717607058636,18.0355031018739,
-21.9858550682355));
#100521=CARTESIAN_POINT('Ctrl Pts',(-17.0143920255779,17.9739806203857,
-21.9903451714393));
#100522=CARTESIAN_POINT('Ctrl Pts',(-17.0601229488358,17.9149195173194,
-21.994835274643));
#100523=CARTESIAN_POINT('Ctrl Pts',(-17.0776568931743,17.8922745755608,
-21.996556849762));
#100524=CARTESIAN_POINT('Ctrl Pts',(-17.0956460703827,17.8699911414134,
-21.998278424881));
#100525=CARTESIAN_POINT('Ctrl Pts',(-17.1140743056111,17.8480877707428,
-22.));
#100526=CARTESIAN_POINT('',(-20.3539402646795,17.8481050888384,-21.9999997807644));
#100527=CARTESIAN_POINT('Origin',(-18.734,19.211,-22.));
#100528=CARTESIAN_POINT('',(-20.8509997094733,19.2098909057104,-21.2890562790225));
#100529=CARTESIAN_POINT('Ctrl Pts',(-20.3539402646795,17.8481050888384,
-21.9999997807644));
#100530=CARTESIAN_POINT('Ctrl Pts',(-20.3072934957001,17.7926606237751,
-21.9956147707751));
#100531=CARTESIAN_POINT('Ctrl Pts',(-20.2577053013778,17.7395048193498,
-21.9912297607858));
#100532=CARTESIAN_POINT('Ctrl Pts',(-20.2054290597327,17.6889666487971,
-21.9868447507965));
#100533=CARTESIAN_POINT('Ctrl Pts',(-20.1532304392223,17.6385035186453,
-21.982466251785));
#100534=CARTESIAN_POINT('Ctrl Pts',(-20.0983520388586,17.5906506399773,
-21.9780877527736));
#100535=CARTESIAN_POINT('Ctrl Pts',(-20.0410869968869,17.545703455066,-21.9737092537621));
#100536=CARTESIAN_POINT('Ctrl Pts',(-19.9838893502852,17.5008091686081,
-21.969335907817));
#100537=CARTESIAN_POINT('Ctrl Pts',(-19.9243110199867,17.4588140795273,
-21.9649625618719));
#100538=CARTESIAN_POINT('Ctrl Pts',(-19.8626801771137,17.4199751375844,
-21.9605892159267));
#100539=CARTESIAN_POINT('Ctrl Pts',(-19.8010883319371,17.381160771474,-21.9562186372717));
#100540=CARTESIAN_POINT('Ctrl Pts',(-19.7374469588082,17.3454988470316,
-21.9518480586166));
#100541=CARTESIAN_POINT('Ctrl Pts',(-19.6721141643387,17.3132036951593,
-21.9474774799615));
#100542=CARTESIAN_POINT('Ctrl Pts',(-19.6068010732891,17.2809182830347,
-21.9431082194094));
#100543=CARTESIAN_POINT('Ctrl Pts',(-19.539798006527,17.2519978415642,-21.9387389588572));
#100544=CARTESIAN_POINT('Ctrl Pts',(-19.4714871908732,17.2266105111904,
-21.934369698305));
#100545=CARTESIAN_POINT('Ctrl Pts',(-19.4031743543433,17.2012224297694,
-21.9300003084946));
#100546=CARTESIAN_POINT('Ctrl Pts',(-19.33355414576,17.1793678332055,-21.9256309186843));
#100547=CARTESIAN_POINT('Ctrl Pts',(-19.2630266691229,17.1611659132123,
-21.9212615288739));
#100548=CARTESIAN_POINT('Ctrl Pts',(-19.1924273973489,17.142945464138,-21.9168876911383));
#100549=CARTESIAN_POINT('Ctrl Pts',(-19.1209194825959,17.1283852352836,
-21.9125138534028));
#100550=CARTESIAN_POINT('Ctrl Pts',(-19.0489151638194,17.1175536931661,
-21.9081400156672));
#100551=CARTESIAN_POINT('Ctrl Pts',(-18.9768710224476,17.1067161605729,
-21.9037637589438));
#100552=CARTESIAN_POINT('Ctrl Pts',(-18.9043304115686,17.0996114670891,
-21.8993875022204));
#100553=CARTESIAN_POINT('Ctrl Pts',(-18.8317099769259,17.096256100515,-21.895011245497));
#100554=CARTESIAN_POINT('Ctrl Pts',(-18.7589654023404,17.0928949981583,
-21.8906275078454));
#100555=CARTESIAN_POINT('Ctrl Pts',(-18.6861412147951,17.0932960158796,
-21.8862437701938));
#100556=CARTESIAN_POINT('Ctrl Pts',(-18.6136526546588,17.0974235248117,
-21.8818600325422));
#100557=CARTESIAN_POINT('Ctrl Pts',(-18.5716446773508,17.099815465019,-21.8793196047637));
#100558=CARTESIAN_POINT('Ctrl Pts',(-18.5297493105789,17.1034579173405,
-21.8767791769852));
#100559=CARTESIAN_POINT('Ctrl Pts',(-18.4880458594114,17.1083360799388,
-21.8742387492067));
#100560=CARTESIAN_POINT('Ctrl Pts',(-18.4158852200683,17.116776900112,-21.8698429764932));
#100561=CARTESIAN_POINT('Ctrl Pts',(-18.3440242584073,17.1289525208195,
-21.8654472037797));
#100562=CARTESIAN_POINT('Ctrl Pts',(-18.272878821027,17.1448305349506,-21.8610514310662));
#100563=CARTESIAN_POINT('Ctrl Pts',(-18.2018362105903,17.160685600489,-21.8566620115904));
#100564=CARTESIAN_POINT('Ctrl Pts',(-18.1315075364803,17.1802323315536,
-21.8522725921145));
#100565=CARTESIAN_POINT('Ctrl Pts',(-18.0623022824371,17.2033866965422,
-21.8478831726387));
#100566=CARTESIAN_POINT('Ctrl Pts',(-17.9931750463637,17.2265149586492,
-21.8434987015386));
#100567=CARTESIAN_POINT('Ctrl Pts',(-17.9251691678202,17.2532426232453,
-21.8391142304384));
#100568=CARTESIAN_POINT('Ctrl Pts',(-17.8586810826102,17.2834352688276,
-21.8347297593383));
#100569=CARTESIAN_POINT('Ctrl Pts',(-17.7922332814893,17.3136096211591,
-21.8303479447205));
#100570=CARTESIAN_POINT('Ctrl Pts',(-17.7273018852858,17.3472445902797,
-21.8259661301027));
#100571=CARTESIAN_POINT('Ctrl Pts',(-17.6642640529712,17.384157367578,-21.8215843154849));
#100572=CARTESIAN_POINT('Ctrl Pts',(-17.601243827434,17.4210598349556,-21.8172037247295));
#100573=CARTESIAN_POINT('Ctrl Pts',(-17.5401165299889,17.4612380500253,
-21.8128231339742));
#100574=CARTESIAN_POINT('Ctrl Pts',(-17.4812339028314,17.5044637109674,
-21.8084425432188));
#100575=CARTESIAN_POINT('Ctrl Pts',(-17.4223484927206,17.547691414872,-21.8040617454248));
#100576=CARTESIAN_POINT('Ctrl Pts',(-17.365708349646,17.5939665647424,-21.7996809476307));
#100577=CARTESIAN_POINT('Ctrl Pts',(-17.3116341001189,17.6430190540522,
-21.7953001498367));
#100578=CARTESIAN_POINT('Ctrl Pts',(-17.2575027316979,17.692123357746,-21.7909147245846));
#100579=CARTESIAN_POINT('Ctrl Pts',(-17.2059430246541,17.7440105345835,
-21.7865292993325));
#100580=CARTESIAN_POINT('Ctrl Pts',(-17.1572399043858,17.798372447926,-21.7821438740803));
#100581=CARTESIAN_POINT('Ctrl Pts',(-17.1085095392263,17.852764771731,-21.7777559955884));
#100582=CARTESIAN_POINT('Ctrl Pts',(-17.0626392444271,17.9096342143152,
-21.7733681170964));
#100583=CARTESIAN_POINT('Ctrl Pts',(-17.0198729444951,17.9686403750982,
-21.7689802386045));
#100584=CARTESIAN_POINT('Ctrl Pts',(-16.9770309082245,18.0277510319582,
-21.7645845894648));
#100585=CARTESIAN_POINT('Ctrl Pts',(-16.9373041057529,18.0890055601327,
-21.7601889403251));
#100586=CARTESIAN_POINT('Ctrl Pts',(-16.9008922045882,18.1520359730375,
-21.7557932911855));
#100587=CARTESIAN_POINT('Ctrl Pts',(-16.8767858983712,18.1937649238989,
-21.7528831749654));
#100588=CARTESIAN_POINT('Ctrl Pts',(-16.8541315758308,18.2362717295104,
-21.7499730587453));
#100589=CARTESIAN_POINT('Ctrl Pts',(-16.8329755513189,18.2794448242231,
-21.7470629425252));
#100590=CARTESIAN_POINT('Ctrl Pts',(-16.8011149074337,18.3444628334097,
-21.7426803527574));
#100591=CARTESIAN_POINT('Ctrl Pts',(-16.772529978103,18.4112473176336,-21.7382977629896));
#100592=CARTESIAN_POINT('Ctrl Pts',(-16.7474198249775,18.4794344129146,
-21.7339151732219));
#100593=CARTESIAN_POINT('Ctrl Pts',(-16.7223474511024,18.5475189179272,
-21.7295391772393));
#100594=CARTESIAN_POINT('Ctrl Pts',(-16.7007396419766,18.6170013950868,
-21.7251631812567));
#100595=CARTESIAN_POINT('Ctrl Pts',(-16.6827487806458,18.6874950476855,
-21.7207871852741));
#100596=CARTESIAN_POINT('Ctrl Pts',(-16.6647794728902,18.7579042468375,
-21.7164164318621));
#100597=CARTESIAN_POINT('Ctrl Pts',(-16.650418624554,18.8293217487381,-21.71204567845));
#100598=CARTESIAN_POINT('Ctrl Pts',(-16.6397692918518,18.9013441570891,
-21.7076749250379));
#100599=CARTESIAN_POINT('Ctrl Pts',(-16.6291268554032,18.973319925447,-21.7033070020215));
#100600=CARTESIAN_POINT('Ctrl Pts',(-16.6221912368165,19.0458993457387,
-21.698939079005));
#100601=CARTESIAN_POINT('Ctrl Pts',(-16.6190144349639,19.1186687502037,
-21.6945711559885));
#100602=CARTESIAN_POINT('Ctrl Pts',(-16.6158386349475,19.19141520611,-21.6902046104402));
#100603=CARTESIAN_POINT('Ctrl Pts',(-16.6164193196609,19.2643510442235,
-21.6858380648919));
#100604=CARTESIAN_POINT('Ctrl Pts',(-16.6207564965869,19.3370590944058,
-21.6814715193436));
#100605=CARTESIAN_POINT('Ctrl Pts',(-16.6250937465921,19.4097683696811,
-21.6771049002213));
#100606=CARTESIAN_POINT('Ctrl Pts',(-16.6331875836567,19.4822493665785,
-21.6727382810989));
#100607=CARTESIAN_POINT('Ctrl Pts',(-16.6449860089037,19.5540882466713,
-21.6683716619766));
#100608=CARTESIAN_POINT('Ctrl Pts',(-16.6567966463011,19.6260014847561,
-21.6640005231147));
#100609=CARTESIAN_POINT('Ctrl Pts',(-16.6723194491993,19.6972708005986,
-21.6596293842528));
#100610=CARTESIAN_POINT('Ctrl Pts',(-16.6914510872628,19.7674916343271,
-21.6552582453909));
#100611=CARTESIAN_POINT('Ctrl Pts',(-16.7105931022024,19.8377505553794,
-21.6508847356516));
#100612=CARTESIAN_POINT('Ctrl Pts',(-16.7333476979536,19.9069594022358,
-21.6465112259124));
#100613=CARTESIAN_POINT('Ctrl Pts',(-16.7595621821267,19.9747305174941,
-21.6421377161732));
#100614=CARTESIAN_POINT('Ctrl Pts',(-16.7858234022015,20.0426224569562,
-21.6377564092208));
#100615=CARTESIAN_POINT('Ctrl Pts',(-16.8155566307479,20.1090711042367,
-21.6333751022684));
#100616=CARTESIAN_POINT('Ctrl Pts',(-16.8485619796008,20.1737110008893,
-21.6289937953161));
#100617=CARTESIAN_POINT('Ctrl Pts',(-16.8714294691446,20.2184962315317,
-21.6259582421587));
#100618=CARTESIAN_POINT('Ctrl Pts',(-16.8958666987907,20.2624137158362,
-21.6229226890013));
#100619=CARTESIAN_POINT('Ctrl Pts',(-16.9217951496002,20.3053503004923,
-21.6198871358439));
#100620=CARTESIAN_POINT('Ctrl Pts',(-16.9592870711159,20.3674355779312,
-21.6154977983717));
#100621=CARTESIAN_POINT('Ctrl Pts',(-17.0000461372983,20.4277127259959,
-21.6111084608995));
#100622=CARTESIAN_POINT('Ctrl Pts',(-17.0438725612033,20.4858169439674,
-21.6067191234274));
#100623=CARTESIAN_POINT('Ctrl Pts',(-17.0876339985392,20.5438350040133,
-21.6023362945397));
#100624=CARTESIAN_POINT('Ctrl Pts',(-17.1344534764691,20.5996861485813,
-21.597953465652));
#100625=CARTESIAN_POINT('Ctrl Pts',(-17.1840867418393,20.6530325558661,
-21.5935706367643));
#100626=CARTESIAN_POINT('Ctrl Pts',(-17.2336617074652,20.7063163019118,
-21.5891929559925));
#100627=CARTESIAN_POINT('Ctrl Pts',(-17.2860435680415,20.7571008040507,
-21.5848152752207));
#100628=CARTESIAN_POINT('Ctrl Pts',(-17.3409474964239,20.8050808393179,
-21.580437594449));
#100629=CARTESIAN_POINT('Ctrl Pts',(-17.3958166125325,20.853030452461,-21.5760626893806));
#100630=CARTESIAN_POINT('Ctrl Pts',(-17.4532042613681,20.8981788105171,
-21.5716877843123));
#100631=CARTESIAN_POINT('Ctrl Pts',(-17.512789428658,20.9402581474269,-21.5673128792439));
#100632=CARTESIAN_POINT('Ctrl Pts',(-17.5723564435283,20.9823246650092,
-21.5629393069756));
#100633=CARTESIAN_POINT('Ctrl Pts',(-17.6341192541722,21.0213237397462,
-21.5585657347073));
#100634=CARTESIAN_POINT('Ctrl Pts',(-17.6977258376919,21.0570294852826,
-21.5541921624389));
#100635=CARTESIAN_POINT('Ctrl Pts',(-17.7613339958298,21.0927361147356,
-21.5498184819002));
#100636=CARTESIAN_POINT('Ctrl Pts',(-17.826785596102,21.1251490188774,-21.5454448013616));
#100637=CARTESIAN_POINT('Ctrl Pts',(-17.8937033322731,21.1540878802069,
-21.5410711208229));
#100638=CARTESIAN_POINT('Ctrl Pts',(-17.9606902956987,21.1830566791589,
-21.5366929156557));
#100639=CARTESIAN_POINT('Ctrl Pts',(-18.0291459798704,21.2085440679544,
-21.5323147104885));
#100640=CARTESIAN_POINT('Ctrl Pts',(-18.0986731480005,21.2304179337444,
-21.5279365053214));
#100641=CARTESIAN_POINT('Ctrl Pts',(-18.1682381862999,21.2523037138266,
-21.5235559154264));
#100642=CARTESIAN_POINT('Ctrl Pts',(-18.2388754035045,21.2705719312819,
-21.5191753255314));
#100643=CARTESIAN_POINT('Ctrl Pts',(-18.3101750846391,21.2851411333656,
-21.5147947356365));
#100644=CARTESIAN_POINT('Ctrl Pts',(-18.3816007583693,21.2997360804675,
-21.5104064048669));
#100645=CARTESIAN_POINT('Ctrl Pts',(-18.4536907566283,21.3106188870059,
-21.5060180740973));
#100646=CARTESIAN_POINT('Ctrl Pts',(-18.5260285057222,21.3177598006341,
-21.5016297433277));
#100647=CARTESIAN_POINT('Ctrl Pts',(-18.5750325606489,21.3225972987322,
-21.4986569386059));
#100648=CARTESIAN_POINT('Ctrl Pts',(-18.6241502208557,21.3257186676998,
-21.4956841338842));
#100649=CARTESIAN_POINT('Ctrl Pts',(-18.6732524671973,21.3271282421579,
-21.4927113291624));
#100650=CARTESIAN_POINT('Ctrl Pts',(-18.7457477304191,21.3292093581758,
-21.4883222374839));
#100651=CARTESIAN_POINT('Ctrl Pts',(-18.8184908959863,21.3275648466035,
-21.4839331458055));
#100652=CARTESIAN_POINT('Ctrl Pts',(-18.8910671061329,21.3221653000585,
-21.479544054127));
#100653=CARTESIAN_POINT('Ctrl Pts',(-18.963535950148,21.316773741371,-21.4751614554825));
#100654=CARTESIAN_POINT('Ctrl Pts',(-19.0358378521743,21.3076382108716,
-21.4707788568379));
#100655=CARTESIAN_POINT('Ctrl Pts',(-19.1075565804155,21.2947812940009,
-21.4663962581934));
#100656=CARTESIAN_POINT('Ctrl Pts',(-19.1791914639276,21.2819394078585,
-21.462018783145));
#100657=CARTESIAN_POINT('Ctrl Pts',(-19.2502440557651,21.2653848625367,
-21.4576413080965));
#100658=CARTESIAN_POINT('Ctrl Pts',(-19.3203035805937,21.2451920045519,
-21.4532638330481));
#100659=CARTESIAN_POINT('Ctrl Pts',(-19.3903189251763,21.2250118803879,
-21.4488891184798));
#100660=CARTESIAN_POINT('Ctrl Pts',(-19.4593419831432,21.2011981291416,
-21.4445144039115));
#100661=CARTESIAN_POINT('Ctrl Pts',(-19.526973898285,21.1738757975579,-21.4401396893431));
#100662=CARTESIAN_POINT('Ctrl Pts',(-19.5945854490438,21.1465616928953,
-21.4357662920281));
#100663=CARTESIAN_POINT('Ctrl Pts',(-19.6608062418169,21.1157412858173,
-21.4313928947131));
#100664=CARTESIAN_POINT('Ctrl Pts',(-19.7252558616823,21.0815883610994,
-21.427019497398));
#100665=CARTESIAN_POINT('Ctrl Pts',(-19.789707311205,21.0474344668157,-21.4226459759268));
#100666=CARTESIAN_POINT('Ctrl Pts',(-19.8523870628951,21.0099480945831,
-21.4182724544556));
#100667=CARTESIAN_POINT('Ctrl Pts',(-19.9129393440595,20.9693489480272,
-21.4138989329844));
#100668=CARTESIAN_POINT('Ctrl Pts',(-19.9735546264145,20.9287075603779,
-21.4095208611139));
#100669=CARTESIAN_POINT('Ctrl Pts',(-20.0320376175175,20.8849472013051,
-21.4051427892433));
#100670=CARTESIAN_POINT('Ctrl Pts',(-20.0880622982484,20.8383304189569,
-21.4007647173728));
#100671=CARTESIAN_POINT('Ctrl Pts',(-20.1441176775264,20.7916880930898,
-21.3963842465516));
#100672=CARTESIAN_POINT('Ctrl Pts',(-20.1977117100798,20.7421865550631,
-21.3920037757304));
#100673=CARTESIAN_POINT('Ctrl Pts',(-20.2485542308314,20.6901262562305,
-21.3876233049092));
#100674=CARTESIAN_POINT('Ctrl Pts',(-20.2994868807634,20.637973669447,-21.3832350687719));
#100675=CARTESIAN_POINT('Ctrl Pts',(-20.3476579595778,20.5832536259681,
-21.3788468326346));
#100676=CARTESIAN_POINT('Ctrl Pts',(-20.3928170701037,20.5263003185328,
-21.3744585964973));
#100677=CARTESIAN_POINT('Ctrl Pts',(-20.4234260340952,20.4876972168292,
-21.3714842384918));
#100678=CARTESIAN_POINT('Ctrl Pts',(-20.4526521165782,20.448068783469,-21.3685098804864));
#100679=CARTESIAN_POINT('Ctrl Pts',(-20.4804290561878,20.407526034695,-21.3655355224809));
#100680=CARTESIAN_POINT('Ctrl Pts',(-20.5219871935396,20.3468684840126,
-21.361085472178));
#100681=CARTESIAN_POINT('Ctrl Pts',(-20.5604590169179,20.2839304044478,
-21.356635421875));
#100682=CARTESIAN_POINT('Ctrl Pts',(-20.5955899436348,20.2190535113564,
-21.3521853715721));
#100683=CARTESIAN_POINT('Ctrl Pts',(-20.6306645775744,20.1542805751153,
-21.3477424519006));
#100684=CARTESIAN_POINT('Ctrl Pts',(-20.6624087272335,20.0875754000713,
-21.3432995322291));
#100685=CARTESIAN_POINT('Ctrl Pts',(-20.6906107246637,20.0193090201965,
-21.3388566125576));
#100686=CARTESIAN_POINT('Ctrl Pts',(-20.7187694166618,19.9511474664102,
-21.3344205151885));
#100687=CARTESIAN_POINT('Ctrl Pts',(-20.7433965961624,19.8814299018275,
-21.3299844178194));
#100688=CARTESIAN_POINT('Ctrl Pts',(-20.7643270348899,19.8105507746598,
-21.3255483204504));
#100689=CARTESIAN_POINT('Ctrl Pts',(-20.7852384845802,19.7397359522305,
-21.3211162477088));
#100690=CARTESIAN_POINT('Ctrl Pts',(-20.8024597234804,19.667762104018,-21.3166841749672));
#100691=CARTESIAN_POINT('Ctrl Pts',(-20.8158744345335,19.5950414545796,
-21.3122521022256));
#100692=CARTESIAN_POINT('Ctrl Pts',(-20.8292816033587,19.5223616912788,
-21.307822521353));
#100693=CARTESIAN_POINT('Ctrl Pts',(-20.8388864096936,19.4489364165862,
-21.3033929404804));
#100694=CARTESIAN_POINT('Ctrl Pts',(-20.8446233306527,19.3751893909619,
-21.2989633596079));
#100695=CARTESIAN_POINT('Ctrl Pts',(-20.8489003446554,19.3202091910428,
-21.2956609994128));
#100696=CARTESIAN_POINT('Ctrl Pts',(-20.8510286075112,19.2650504520942,
-21.2923586392176));
#100697=CARTESIAN_POINT('Ctrl Pts',(-20.8509997094733,19.2098909057104,
-21.2890562790225));
#100698=CARTESIAN_POINT('Ctrl Pts',(-20.8509997571968,19.2099860824115,
-21.2873808744862));
#100699=CARTESIAN_POINT('Ctrl Pts',(-20.8509646300435,19.1366426709241,
-21.2832143337499));
#100700=CARTESIAN_POINT('Ctrl Pts',(-20.8471180797899,19.0633455484618,
-21.279152411229));
#100701=CARTESIAN_POINT('Ctrl Pts',(-20.8225239542534,18.828621677677,-21.2662357234474));
#100702=CARTESIAN_POINT('Ctrl Pts',(-20.7869893936289,18.6693653068234,
-21.2576412236419));
#100703=CARTESIAN_POINT('Ctrl Pts',(-20.729996333494,18.5054455806247,-21.2476752856251));
#100704=CARTESIAN_POINT('Ctrl Pts',(-20.7263281350187,18.4951529628947,
-21.2470444477784));
#100705=CARTESIAN_POINT('Ctrl Pts',(-20.7225806138391,18.4848897175613,
-21.2464098975766));
#100706=CARTESIAN_POINT('Origin',(-18.734,19.211,0.));
#100707=CARTESIAN_POINT('',(-20.7225807433525,18.4848900722565,-20.4442393203449));
#100708=CARTESIAN_POINT('',(-20.7225806137969,18.4848897174457,-20.6683679590049));
#100709=CARTESIAN_POINT('',(-20.7225806137986,18.4848897174502,0.));
#100710=CARTESIAN_POINT('Ctrl Pts',(-20.7225806137969,18.4848897174457,
-20.6683679590049));
#100711=CARTESIAN_POINT('Ctrl Pts',(-20.7238652346132,18.4884078773075,
-20.6685903986784));
#100712=CARTESIAN_POINT('Ctrl Pts',(-20.7251405258313,18.4919294648717,
-20.6688125292484));
#100713=CARTESIAN_POINT('Ctrl Pts',(-20.7310458686688,18.5083726433526,
-20.6698472828421));
#100714=CARTESIAN_POINT('Ctrl Pts',(-20.7355595959726,18.5213358782087,
-20.6706560544971));
#100715=CARTESIAN_POINT('Ctrl Pts',(-20.7688588121525,18.6200511751937,
-20.6767638173075));
#100716=CARTESIAN_POINT('Ctrl Pts',(-20.7922497953967,18.7075304791077,
-20.6818795084204));
#100717=CARTESIAN_POINT('Ctrl Pts',(-20.8373639114506,18.9333413712789,
-20.6946257510643));
#100718=CARTESIAN_POINT('Ctrl Pts',(-20.8511051845657,19.0728052824219,
-20.7020608117507));
#100719=CARTESIAN_POINT('Ctrl Pts',(-20.8509840406739,19.2328904078365,
-20.7109057277407));
#100720=CARTESIAN_POINT('Ctrl Pts',(-20.8506770362226,19.253177132247,-20.7120328020567));
#100721=CARTESIAN_POINT('Ctrl Pts',(-20.8483264321579,19.332818346702,-20.7164920697114));
#100722=CARTESIAN_POINT('Ctrl Pts',(-20.8440773388105,19.3920752179361,
-20.7198853164855));
#100723=CARTESIAN_POINT('Ctrl Pts',(-20.8363297205134,19.459955297946,-20.7239378705037));
#100724=CARTESIAN_POINT('Ctrl Pts',(-20.8352591881887,19.4688348537521,
-20.7244712782586));
#100725=CARTESIAN_POINT('Ctrl Pts',(-20.8335616373004,19.4822018792377,
-20.7252795633576));
#100726=CARTESIAN_POINT('Ctrl Pts',(-20.8329764095954,19.4866946847716,
-20.725552141968));
#100727=CARTESIAN_POINT('Ctrl Pts',(-20.8319046586591,19.4947212851328,
-20.7260407894413));
#100728=CARTESIAN_POINT('Ctrl Pts',(-20.8314236226012,19.4982557598237,
-20.7262565460338));
#100729=CARTESIAN_POINT('Ctrl Pts',(-20.8303644473523,19.5058936686,-20.7267240650099));
#100730=CARTESIAN_POINT('Ctrl Pts',(-20.8297832003999,19.5099965687839,
-20.7269759956357));
#100731=CARTESIAN_POINT('Ctrl Pts',(-20.8281309514489,19.5214178873796,
-20.7276794520146));
#100732=CARTESIAN_POINT('Ctrl Pts',(-20.8270336482833,19.5287323560194,
-20.7281324246829));
#100733=CARTESIAN_POINT('Ctrl Pts',(-20.8205389580125,19.5705308933003,
-20.7307344515959));
#100734=CARTESIAN_POINT('Ctrl Pts',(-20.81432804568,19.6048809225384,-20.732925408145));
#100735=CARTESIAN_POINT('Ctrl Pts',(-20.7918958094138,19.713529682705,-20.739990378814));
#100736=CARTESIAN_POINT('Ctrl Pts',(-20.7725200156514,19.7871126711618,
-20.744976017493));
#100737=CARTESIAN_POINT('Ctrl Pts',(-20.6904215892157,20.0422401707648,
-20.7626582236558));
#100738=CARTESIAN_POINT('Ctrl Pts',(-20.6070117016007,20.2161882405814,
-20.7753361389334));
#100739=CARTESIAN_POINT('Ctrl Pts',(-20.4894886988923,20.3943877308854,
-20.7884543995998));
#100740=CARTESIAN_POINT('Ctrl Pts',(-20.477434543749,20.4120758252533,-20.7897596208203));
#100741=CARTESIAN_POINT('Ctrl Pts',(-20.4603099695348,20.4364030108672,
-20.7915596757558));
#100742=CARTESIAN_POINT('Ctrl Pts',(-20.4554657132109,20.4431990307239,
-20.792063084789));
#100743=CARTESIAN_POINT('Ctrl Pts',(-20.4470415409645,20.454870677359,-20.7929286584956));
#100744=CARTESIAN_POINT('Ctrl Pts',(-20.4434807113584,20.4597598975535,
-20.7932915529839));
#100745=CARTESIAN_POINT('Ctrl Pts',(-20.4360700412671,20.4698440656833,
-20.794040704147));
#100746=CARTESIAN_POINT('Ctrl Pts',(-20.4322172523278,20.4750367765269,
-20.7944268409867));
#100747=CARTESIAN_POINT('Ctrl Pts',(-20.4231497182478,20.4871415269331,
-20.7953278842125));
#100748=CARTESIAN_POINT('Ctrl Pts',(-20.417916214374,20.494039420199,-20.7958420496878));
#100749=CARTESIAN_POINT('Ctrl Pts',(-20.4008334149364,20.5162704190809,
-20.7975016064568));
#100750=CARTESIAN_POINT('Ctrl Pts',(-20.3888156628372,20.5314732708375,
-20.7986403352536));
#100751=CARTESIAN_POINT('Ctrl Pts',(-20.3265598481577,20.6080439164203,
-20.8043989788289));
#100752=CARTESIAN_POINT('Ctrl Pts',(-20.2731078844067,20.6667223149236,
-20.8088862894284));
#100753=CARTESIAN_POINT('Ctrl Pts',(-20.1000689128619,20.8364655915517,
-20.8223348306495));
#100754=CARTESIAN_POINT('Ctrl Pts',(-19.9708585941075,20.9368208953897,
-20.8309358542029));
#100755=CARTESIAN_POINT('Ctrl Pts',(-19.7791774678144,21.0530166252851,
-20.8434651113487));
#100756=CARTESIAN_POINT('Ctrl Pts',(-19.7255937341235,21.0824063123928,
-20.8469515638519));
#100757=CARTESIAN_POINT('Ctrl Pts',(-19.6626471178312,21.1134685529451,
-20.8511147275503));
#100758=CARTESIAN_POINT('Ctrl Pts',(-19.6544483063012,21.1174487858551,
-20.8516582659053));
#100759=CARTESIAN_POINT('Ctrl Pts',(-19.6421586496759,21.123317223867,-20.8524752965509));
#100760=CARTESIAN_POINT('Ctrl Pts',(-19.6380869386098,21.1252455705193,
-20.8527463620862));
#100761=CARTESIAN_POINT('Ctrl Pts',(-19.6307807916038,21.1286772234577,
-20.8532334758977));
#100762=CARTESIAN_POINT('Ctrl Pts',(-19.6275486861925,21.1301853653746,
-20.853449221096));
#100763=CARTESIAN_POINT('Ctrl Pts',(-19.6205325546384,21.133437616634,-20.8539181167342));
#100764=CARTESIAN_POINT('Ctrl Pts',(-19.6167472360457,21.1351787019003,
-20.8541714431054));
#100765=CARTESIAN_POINT('Ctrl Pts',(-19.6061409439359,21.1400192603131,
-20.8548821771415));
#100766=CARTESIAN_POINT('Ctrl Pts',(-19.5993086988774,21.1430936790285,
-20.8553410773669));
#100767=CARTESIAN_POINT('Ctrl Pts',(-19.5591797901109,21.1608956088416,
-20.8580420257431));
#100768=CARTESIAN_POINT('Ctrl Pts',(-19.525526096485,21.1747975052504,-20.8603296642863));
#100769=CARTESIAN_POINT('Ctrl Pts',(-19.4153876736243,21.2170033453429,
-20.8678506049317));
#100770=CARTESIAN_POINT('Ctrl Pts',(-19.3376246634642,21.2417570242178,
-20.8732107339635));
#100771=CARTESIAN_POINT('Ctrl Pts',(-19.0810913452032,21.3073779395742,
-20.8906948008783));
#100772=CARTESIAN_POINT('Ctrl Pts',(-18.8983629616855,21.3295571239798,
-20.9027594276025));
#100773=CARTESIAN_POINT('Ctrl Pts',(-18.692724428247,21.3277152135146,-20.9154088546417));
#100774=CARTESIAN_POINT('Ctrl Pts',(-18.6704140468334,21.3271625302196,
-20.9167705223312));
#100775=CARTESIAN_POINT('Ctrl Pts',(-18.6396296753637,21.325912616701,-20.9186352215502));
#100776=CARTESIAN_POINT('Ctrl Pts',(-18.6311455225524,21.3255169883947,
-20.9191476478689));
#100777=CARTESIAN_POINT('Ctrl Pts',(-18.6165837343287,21.3247501014288,
-20.9200246650255));
#100778=CARTESIAN_POINT('Ctrl Pts',(-18.6105049471499,21.3244036632551,
-20.920390029593));
#100779=CARTESIAN_POINT('Ctrl Pts',(-18.5979923812975,21.3236363853174,
-20.9211405933597));
#100780=CARTESIAN_POINT('Ctrl Pts',(-18.5915588554447,21.3232123687426,
-20.9215256888571));
#100781=CARTESIAN_POINT('Ctrl Pts',(-18.5766193347189,21.3221591772321,
-20.922418077333));
#100782=CARTESIAN_POINT('Ctrl Pts',(-18.5681149671147,21.3215079731021,
-20.9229246736432));
#100783=CARTESIAN_POINT('Ctrl Pts',(-18.5410182405817,21.3192683013282,
-20.9245344989172));
#100784=CARTESIAN_POINT('Ctrl Pts',(-18.5224425239929,21.3174853802474,
-20.9256316224427));
#100785=CARTESIAN_POINT('Ctrl Pts',(-18.3441712716333,21.2979926669864,
-20.9361045577907));
#100786=CARTESIAN_POINT('Ctrl Pts',(-18.186954372689,21.2624029531223,-20.9448518902129));
#100787=CARTESIAN_POINT('Ctrl Pts',(-17.908489805109,21.1650362875258,-20.9608716365759));
#100788=CARTESIAN_POINT('Ctrl Pts',(-17.7862406205074,21.1087531818223,
-20.9681341966779));
#100789=CARTESIAN_POINT('Ctrl Pts',(-17.6566075194641,21.0334050827816,
-20.9769255641358));
#100790=CARTESIAN_POINT('Ctrl Pts',(-17.6431400772507,21.0253757712625,
-20.9778530778051));
#100791=CARTESIAN_POINT('Ctrl Pts',(-17.6248244002669,21.0141783055513,
-20.9791357969203));
#100792=CARTESIAN_POINT('Ctrl Pts',(-17.6198977606776,21.0111385255583,
-20.9794829645817));
#100793=CARTESIAN_POINT('Ctrl Pts',(-17.6120881042092,21.0062755592598,
-20.9800367960227));
#100794=CARTESIAN_POINT('Ctrl Pts',(-17.6091968773176,21.0044655197175,
-20.9802425986771));
#100795=CARTESIAN_POINT('Ctrl Pts',(-17.6032369892519,21.0007142784723,
-20.9806684486323));
#100796=CARTESIAN_POINT('Ctrl Pts',(-17.600168955563,20.9987721742235,-20.9808885589073));
#100797=CARTESIAN_POINT('Ctrl Pts',(-17.5928703093444,20.9941256941398,
-20.9814142901131));
#100798=CARTESIAN_POINT('Ctrl Pts',(-17.5886443072106,20.9914141506399,
-20.9817203841157));
#100799=CARTESIAN_POINT('Ctrl Pts',(-17.57442015286,20.9822158591705,-20.9827562590519));
#100800=CARTESIAN_POINT('Ctrl Pts',(-17.5644673557949,20.9756598598023,
-20.983490451711));
#100801=CARTESIAN_POINT('Ctrl Pts',(-17.540688908616,20.9597072588907,-20.9852661645549));
#100802=CARTESIAN_POINT('Ctrl Pts',(-17.526918352114,20.950230374788,-20.9863123308712));
#100803=CARTESIAN_POINT('Ctrl Pts',(-17.4756938282233,20.9140763361337,
-20.9902669930896));
#100804=CARTESIAN_POINT('Ctrl Pts',(-17.439001926931,20.8863455983022,-20.993227799718));
#100805=CARTESIAN_POINT('Ctrl Pts',(-17.3454296110854,20.8107148103743,
-21.0010640329972));
#100806=CARTESIAN_POINT('Ctrl Pts',(-17.2901177494593,20.7609737723358,
-21.0059872623381));
#100807=CARTESIAN_POINT('Ctrl Pts',(-17.1277324302756,20.5986932500524,
-21.0211541477343));
#100808=CARTESIAN_POINT('Ctrl Pts',(-17.0303110719726,20.4771945623109,
-21.0312703118379));
#100809=CARTESIAN_POINT('Ctrl Pts',(-16.9342094177865,20.3259062394142,
-21.0423125676483));
#100810=CARTESIAN_POINT('Ctrl Pts',(-16.9217170001419,20.3054827384802,
-21.0437748245359));
#100811=CARTESIAN_POINT('Ctrl Pts',(-16.9046536700756,20.2764928750974,
-21.0458116546682));
#100812=CARTESIAN_POINT('Ctrl Pts',(-16.899791504457,20.2681008757307,-21.0463968010334));
#100813=CARTESIAN_POINT('Ctrl Pts',(-16.8920195799322,20.2544716192993,
-21.0473399979026));
#100814=CARTESIAN_POINT('Ctrl Pts',(-16.8890741224234,20.2492549761941,
-21.0476993358021));
#100815=CARTESIAN_POINT('Ctrl Pts',(-16.8829818648259,20.2383573078666,
-21.0484465497037));
#100816=CARTESIAN_POINT('Ctrl Pts',(-16.8798389788568,20.2326741573979,
-21.0488342821771));
#100817=CARTESIAN_POINT('Ctrl Pts',(-16.8724721085011,20.2192069924331,
-21.0497485508298));
#100818=CARTESIAN_POINT('Ctrl Pts',(-16.8682706978415,20.2114107182159,
-21.0502742766826));
#100819=CARTESIAN_POINT('Ctrl Pts',(-16.8544955238803,20.1854604344387,
-21.0520126238802));
#100820=CARTESIAN_POINT('Ctrl Pts',(-16.8451366468869,20.1671932289247,
-21.0532176403368));
#100821=CARTESIAN_POINT('Ctrl Pts',(-16.7969196933668,20.06960912344,-21.0595612073592));
#100822=CARTESIAN_POINT('Ctrl Pts',(-16.762785859985,19.9880502692792,-21.0645332885322));
#100823=CARTESIAN_POINT('Ctrl Pts',(-16.6909611660007,19.7809240624421,
-21.076633940842));
#100824=CARTESIAN_POINT('Ctrl Pts',(-16.6596407171892,19.6535530519481,
-21.0836113184103));
#100825=CARTESIAN_POINT('Ctrl Pts',(-16.6347043027225,19.4868063465345,
-21.0929114939677));
#100826=CARTESIAN_POINT('Ctrl Pts',(-16.6301239880343,19.4493632957288,
-21.0950118496028));
#100827=CARTESIAN_POINT('Ctrl Pts',(-16.6221952111272,19.3661565949755,
-21.0997432653302));
#100828=CARTESIAN_POINT('Ctrl Pts',(-16.6193295724543,19.3203679203164,
-21.102389568849));
#100829=CARTESIAN_POINT('Ctrl Pts',(-16.6177244757135,19.2669024109276,
-21.1055661136472));
#100830=CARTESIAN_POINT('Ctrl Pts',(-16.6175368076586,19.2592775904332,
-21.1060211791667));
#100831=CARTESIAN_POINT('Ctrl Pts',(-16.6173018816819,19.2470458197098,
-21.1067547253886));
#100832=CARTESIAN_POINT('Ctrl Pts',(-16.6172284509348,19.2424393600136,
-21.1070317798662));
#100833=CARTESIAN_POINT('Ctrl Pts',(-16.6171246650432,19.234251712285,-21.1075257080918));
#100834=CARTESIAN_POINT('Ctrl Pts',(-16.6170883600617,19.2306706475776,
-21.1077422458778));
#100835=CARTESIAN_POINT('Ctrl Pts',(-16.6170304170128,19.2230469031411,
-21.1082043308926));
#100836=CARTESIAN_POINT('Ctrl Pts',(-16.6170112722208,19.2190043107715,
-21.1084500090353));
#100837=CARTESIAN_POINT('Ctrl Pts',(-16.6169907239663,19.2080241066514,
-21.1091190261681));
#100838=CARTESIAN_POINT('Ctrl Pts',(-16.6170118442319,19.2010865741262,
-21.1095435945458));
#100839=CARTESIAN_POINT('Ctrl Pts',(-16.6172932400599,19.1657349853193,
-21.1117161605605));
#100840=CARTESIAN_POINT('Ctrl Pts',(-16.618091467561,19.1373296005919,-21.1134917535019));
#100841=CARTESIAN_POINT('Ctrl Pts',(-16.6221164440865,19.0539291421224,
-21.1187764209565));
#100842=CARTESIAN_POINT('Ctrl Pts',(-16.6269181780206,18.9990359186557,
-21.1223457032781));
#100843=CARTESIAN_POINT('Ctrl Pts',(-16.6514754102595,18.8055884773547,
-21.1351165688919));
#100844=CARTESIAN_POINT('Ctrl Pts',(-16.6828169386274,18.6688559358138,
-21.1444680068812));
#100845=CARTESIAN_POINT('Ctrl Pts',(-16.7562388452252,18.4505243812992,
-21.1593417237258));
#100846=CARTESIAN_POINT('Ctrl Pts',(-16.7905178048905,18.3667588904991,
-21.1650403449655));
#100847=CARTESIAN_POINT('Ctrl Pts',(-16.8360573533758,18.273081400192,-21.1713958568454));
#100848=CARTESIAN_POINT('Ctrl Pts',(-16.8421815755244,18.2607891536605,
-21.1722296015031));
#100849=CARTESIAN_POINT('Ctrl Pts',(-16.8521958699974,18.2411695968639,
-21.1735601876361));
#100850=CARTESIAN_POINT('Ctrl Pts',(-16.8560100733402,18.2338041992708,
-21.1740596714804));
#100851=CARTESIAN_POINT('Ctrl Pts',(-16.8628598094688,18.2207652873705,
-21.1749439080675));
#100852=CARTESIAN_POINT('Ctrl Pts',(-16.8658780886411,18.2150828727072,
-21.1753292636354));
#100853=CARTESIAN_POINT('Ctrl Pts',(-16.8722213227627,18.2032709785249,
-21.1761303343288));
#100854=CARTESIAN_POINT('Ctrl Pts',(-16.8755507543537,18.1971439811875,
-21.1765458845793));
#100855=CARTESIAN_POINT('Ctrl Pts',(-16.8842770147452,18.1812728771118,
-21.1776224368516));
#100856=CARTESIAN_POINT('Ctrl Pts',(-16.8897206261015,18.1715546344465,
-21.1782817610144));
#100857=CARTESIAN_POINT('Ctrl Pts',(-16.9137061157043,18.1295160435795,
-21.1811349016419));
#100858=CARTESIAN_POINT('Ctrl Pts',(-16.9330234362541,18.0976442438993,
-21.1833006497502));
#100859=CARTESIAN_POINT('Ctrl Pts',(-16.9865976085496,18.0142982800807,
-21.1889869011616));
#100860=CARTESIAN_POINT('Ctrl Pts',(-17.0222853097246,17.9637855831186,
-21.1924562585561));
#100861=CARTESIAN_POINT('Ctrl Pts',(-17.1467844133524,17.8029990871616,
-21.2037070626936));
#100862=CARTESIAN_POINT('Ctrl Pts',(-17.244432781696,17.7000707935218,-21.2112299041505));
#100863=CARTESIAN_POINT('Ctrl Pts',(-17.4090248353282,17.5581614134058,
-21.2232601561996));
#100864=CARTESIAN_POINT('Ctrl Pts',(-17.4690435227198,17.5117892711482,
-21.2275427149157));
#100865=CARTESIAN_POINT('Ctrl Pts',(-17.539237091923,17.4633384159903,-21.2325974879184));
#100866=CARTESIAN_POINT('Ctrl Pts',(-17.5470988982186,17.4579896789482,
-21.2331642649796));
#100867=CARTESIAN_POINT('Ctrl Pts',(-17.5588060741698,17.4501396202669,
-21.234009622133));
#100868=CARTESIAN_POINT('Ctrl Pts',(-17.5626240952516,17.4475974568778,
-21.2342855277687));
#100869=CARTESIAN_POINT('Ctrl Pts',(-17.5694372858565,17.4430929020754,
-21.2347783105935));
#100870=CARTESIAN_POINT('Ctrl Pts',(-17.5724291996125,17.4411256831499,
-21.2349948599685));
#100871=CARTESIAN_POINT('Ctrl Pts',(-17.5788817139648,17.43690648726,-21.2354622172894));
#100872=CARTESIAN_POINT('Ctrl Pts',(-17.582343871688,17.4346570691078,-21.2357131842254));
#100873=CARTESIAN_POINT('Ctrl Pts',(-17.5919271525371,17.4284704543625,
-21.236408370159));
#100874=CARTESIAN_POINT('Ctrl Pts',(-17.5980619658802,17.4245547170155,
-21.236853968528));
#100875=CARTESIAN_POINT('Ctrl Pts',(-17.6319353181023,17.4031790140468,
-21.2393169275164));
#100876=CARTESIAN_POINT('Ctrl Pts',(-17.6600546605555,17.3863344374671,
-21.2413709740104));
#100877=CARTESIAN_POINT('Ctrl Pts',(-17.8308695867514,17.2893258792621,
-21.2538531240551));
#100878=CARTESIAN_POINT('Ctrl Pts',(-17.9820760932208,17.2252792955987,
-21.2648705847584));
#100879=CARTESIAN_POINT('Ctrl Pts',(-18.2489491721557,17.1471434353869,
-21.2830112442204));
#100880=CARTESIAN_POINT('Ctrl Pts',(-18.361186433397,17.1239457147987,-21.2902910156378));
#100881=CARTESIAN_POINT('Ctrl Pts',(-18.488924710063,17.1081850669349,-21.2981493541542));
#100882=CARTESIAN_POINT('Ctrl Pts',(-18.5031016629,17.1065811933026,-21.2990159238424));
#100883=CARTESIAN_POINT('Ctrl Pts',(-18.5257080644195,17.1042548765083,
-21.3003890824671));
#100884=CARTESIAN_POINT('Ctrl Pts',(-18.5341273126123,17.1034394533356,
-21.3008985760084));
#100885=CARTESIAN_POINT('Ctrl Pts',(-18.5489948411865,17.1020893919952,
-21.3017949870334));
#100886=CARTESIAN_POINT('Ctrl Pts',(-18.5554410671652,17.1015338186437,
-21.3021825566988));
#100887=CARTESIAN_POINT('Ctrl Pts',(-18.5687893026233,17.1004450148337,
-21.3029828742049));
#100888=CARTESIAN_POINT('Ctrl Pts',(-18.575691591258,17.0999160676548,-21.3033954832756));
#100889=CARTESIAN_POINT('Ctrl Pts',(-18.5934369133651,17.0986436997339,
-21.3044531783063));
#100890=CARTESIAN_POINT('Ctrl Pts',(-18.6042833867069,17.0979498994373,
-21.3050967049058));
#100891=CARTESIAN_POINT('Ctrl Pts',(-18.6497613108504,17.0953923745097,
-21.3077829610856));
#100892=CARTESIAN_POINT('Ctrl Pts',(-18.6844317031404,17.0942962020218,
-21.3098016555644));
#100893=CARTESIAN_POINT('Ctrl Pts',(-18.7749971765672,17.0936594007023,
-21.3150108109381));
#100894=CARTESIAN_POINT('Ctrl Pts',(-18.830875632806,17.0954793165037,-21.3181606736556));
#100895=CARTESIAN_POINT('Ctrl Pts',(-19.0845512127364,17.1138151352687,
-21.3322947409199));
#100896=CARTESIAN_POINT('Ctrl Pts',(-19.2794566076175,17.1558775631409,
-21.3426052583601));
#100897=CARTESIAN_POINT('Ctrl Pts',(-19.4955730150691,17.2354712891762,
-21.3558294172691));
#100898=CARTESIAN_POINT('Ctrl Pts',(-19.5252603478741,17.2471736430862,
-21.3576899717256));
#100899=CARTESIAN_POINT('Ctrl Pts',(-19.5609553935453,17.2621849063027,
-21.3599938957978));
#100900=CARTESIAN_POINT('Ctrl Pts',(-19.5672278349472,17.264858467493,-21.3604012884993));
#100901=CARTESIAN_POINT('Ctrl Pts',(-19.5775390666039,17.2693125059558,
-21.3610753655013));
#100902=CARTESIAN_POINT('Ctrl Pts',(-19.5815854528846,17.2710754188214,
-21.3613410032996));
#100903=CARTESIAN_POINT('Ctrl Pts',(-19.588876396886,17.2742790730214,-21.3618217028382));
#100904=CARTESIAN_POINT('Ctrl Pts',(-19.5921228733818,17.275715334382,-21.3620364884069));
#100905=CARTESIAN_POINT('Ctrl Pts',(-19.5984344687416,17.2785266277539,
-21.3624555260017));
#100906=CARTESIAN_POINT('Ctrl Pts',(-19.6014998841126,17.2799007700566,
-21.3626597155257));
#100907=CARTESIAN_POINT('Ctrl Pts',(-19.6105435276379,17.283980668308,-21.363264075301));
#100908=CARTESIAN_POINT('Ctrl Pts',(-19.616512394334,17.2867069007629,-21.3636654869535));
#100909=CARTESIAN_POINT('Ctrl Pts',(-19.6448684015059,17.2998179610146,
-21.3655841816581));
#100910=CARTESIAN_POINT('Ctrl Pts',(-19.667084469502,17.3105655023873,-21.3671223254333));
#100911=CARTESIAN_POINT('Ctrl Pts',(-19.7292832157982,17.3420090902268,
-21.3715175443288));
#100912=CARTESIAN_POINT('Ctrl Pts',(-19.7687994160794,17.3635949699764,
-21.3744153798857));
#100913=CARTESIAN_POINT('Ctrl Pts',(-19.8895235802651,17.4346299534854,
-21.3835371507064));
#100914=CARTESIAN_POINT('Ctrl Pts',(-19.9681106256475,17.4882998853338,
-21.3898622740666));
#100915=CARTESIAN_POINT('Ctrl Pts',(-20.1606339789982,17.6397358276908,
-21.4060184879364));
#100916=CARTESIAN_POINT('Ctrl Pts',(-20.2682893331312,17.7446685562577,
-21.4156928918988));
#100917=CARTESIAN_POINT('Ctrl Pts',(-20.3729857877411,17.8709946863554,
-21.425708948531));
#100918=CARTESIAN_POINT('Ctrl Pts',(-20.3818932538555,17.8819640741452,
-21.4265670672809));
#100919=CARTESIAN_POINT('Ctrl Pts',(-20.3959064983343,17.8995786384601,
-21.4279268969339));
#100920=CARTESIAN_POINT('Ctrl Pts',(-20.4010836841691,17.9061662213677,
-21.4284314840876));
#100921=CARTESIAN_POINT('Ctrl Pts',(-20.4101516090927,17.9178465471727,
-21.4293192505649));
#100922=CARTESIAN_POINT('Ctrl Pts',(-20.4140585606511,17.9229265147453,
-21.4297030757404));
#100923=CARTESIAN_POINT('Ctrl Pts',(-20.4220973657185,17.9334776761386,
-21.4304956227197));
#100924=CARTESIAN_POINT('Ctrl Pts',(-20.4262258339122,17.9389513637989,
-21.4309042074721));
#100925=CARTESIAN_POINT('Ctrl Pts',(-20.4367661202862,17.9530682243811,
-21.4319514493149));
#100926=CARTESIAN_POINT('Ctrl Pts',(-20.4431388058203,17.9617404747377,
-21.4325885652028));
#100927=CARTESIAN_POINT('Ctrl Pts',(-20.4695468605432,17.9982581275464,
-21.435245908051));
#100928=CARTESIAN_POINT('Ctrl Pts',(-20.488970717365,18.0265407422626,-21.4372424412269));
#100929=CARTESIAN_POINT('Ctrl Pts',(-20.5378440241057,18.1015475541661,
-21.4423912149845));
#100930=CARTESIAN_POINT('Ctrl Pts',(-20.5661683690365,18.1489747118992,
-21.445503583397));
#100931=CARTESIAN_POINT('Ctrl Pts',(-20.6274493266389,18.2613501573442,
-21.4526165474944));
#100932=CARTESIAN_POINT('Ctrl Pts',(-20.658974556634,18.3269984218444,-21.4565793224947));
#100933=CARTESIAN_POINT('Ctrl Pts',(-20.6995931154224,18.4241148417424,
-21.4622948401121));
#100934=CARTESIAN_POINT('Ctrl Pts',(-20.711437453539,18.4543722148084,-21.4640561340388));
#100935=CARTESIAN_POINT('Ctrl Pts',(-20.7225806137704,18.4848897173731,
-21.4658225507677));
#100936=CARTESIAN_POINT('Ctrl Pts',(-20.7225806138391,18.4848897175613,
-21.2464098975766));
#100937=CARTESIAN_POINT('Ctrl Pts',(-20.7152359994648,18.4647752003672,
-21.2451662684389));
#100938=CARTESIAN_POINT('Ctrl Pts',(-20.707586702596,18.4447735039477,-21.2439083812047));
#100939=CARTESIAN_POINT('Ctrl Pts',(-20.6969531989406,18.4181848178665,
-21.2422033325788));
#100940=CARTESIAN_POINT('Ctrl Pts',(-20.6942367444667,18.4114919784822,
-21.2417713244391));
#100941=CARTESIAN_POINT('Ctrl Pts',(-20.6899234875745,18.4010190441321,
-21.2410906959478));
#100942=CARTESIAN_POINT('Ctrl Pts',(-20.6883498252307,18.3972293946838,
-21.2408434557225));
#100943=CARTESIAN_POINT('Ctrl Pts',(-20.6853860462295,18.3901502868224,
-21.2403797795697));
#100944=CARTESIAN_POINT('Ctrl Pts',(-20.6839986202765,18.3868597611576,
-21.2401635072466));
#100945=CARTESIAN_POINT('Ctrl Pts',(-20.6808109679336,18.3793527945521,
-21.2396684128177));
#100946=CARTESIAN_POINT('Ctrl Pts',(-20.6790053702831,18.3751386910184,
-21.239389266955));
#100947=CARTESIAN_POINT('Ctrl Pts',(-20.6734104194994,18.3621968676265,
-21.2385283072623));
#100948=CARTESIAN_POINT('Ctrl Pts',(-20.6695759641248,18.3534889434377,
-21.2379438451609));
#100949=CARTESIAN_POINT('Ctrl Pts',(-20.6165875202679,18.2353202223973,
-21.2299450063012));
#100950=CARTESIAN_POINT('Ctrl Pts',(-20.5582778615877,18.1302176834212,
-21.2220507285775));
#100951=CARTESIAN_POINT('Ctrl Pts',(-20.4306977127279,17.9402699446208,
-21.2069341869007));
#100952=CARTESIAN_POINT('Ctrl Pts',(-20.3631210364827,17.8547160587159,
-21.1997397457768));
#100953=CARTESIAN_POINT('Ctrl Pts',(-20.252301798355,17.7347154429134,-21.1892458908812));
#100954=CARTESIAN_POINT('Ctrl Pts',(-20.2138109877699,17.6961347651446,
-21.1857978963002));
#100955=CARTESIAN_POINT('Ctrl Pts',(-20.1573001305014,17.6437039968266,
-21.1810074796356));
#100956=CARTESIAN_POINT('Ctrl Pts',(-20.1404826770932,17.6285946904318,
-21.1796136224393));
#100957=CARTESIAN_POINT('Ctrl Pts',(-20.1143229067879,17.6058385619071,
-21.1774930207077));
#100958=CARTESIAN_POINT('Ctrl Pts',(-20.1051522240041,17.5979977813365,
-21.1767583171528));
#100959=CARTESIAN_POINT('Ctrl Pts',(-20.0880167126455,17.5835989526179,
-21.1754013999514));
#100960=CARTESIAN_POINT('Ctrl Pts',(-20.0800700521631,17.5770199365629,
-21.1747783384348));
#100961=CARTESIAN_POINT('Ctrl Pts',(-20.06690184825,17.5662792829195,-21.1737559504324));
#100962=CARTESIAN_POINT('Ctrl Pts',(-20.0617082118684,17.56208384689,-21.1733552581288));
#100963=CARTESIAN_POINT('Ctrl Pts',(-20.0514511068144,17.5538780066179,
-21.1725688653188));
#100964=CARTESIAN_POINT('Ctrl Pts',(-20.0463889625842,17.5498660703872,
-21.1721831057767));
#100965=CARTESIAN_POINT('Ctrl Pts',(-20.0346569859217,17.5406551497722,
-21.1712944239702));
#100966=CARTESIAN_POINT('Ctrl Pts',(-20.0279741760687,17.5354728147413,
-21.1707921675384));
#100967=CARTESIAN_POINT('Ctrl Pts',(-20.0099151881518,17.5216410519944,
-21.169445380337));
#100968=CARTESIAN_POINT('Ctrl Pts',(-19.9984820620083,17.5130664464331,
-21.168603789409));
#100969=CARTESIAN_POINT('Ctrl Pts',(-19.8931905239911,17.4357533870795,
-21.1609510811334));
#100970=CARTESIAN_POINT('Ctrl Pts',(-19.7938966826245,17.3747409118555,
-21.1544535643496));
#100971=CARTESIAN_POINT('Ctrl Pts',(-19.5451166395735,17.2488130918211,
-21.1391851304526));
#100972=CARTESIAN_POINT('Ctrl Pts',(-19.3922058557569,17.1923764489089,
-21.1305981481223));
#100973=CARTESIAN_POINT('Ctrl Pts',(-19.2022751842734,17.1461759830774,
-21.1193807164723));
#100974=CARTESIAN_POINT('Ctrl Pts',(-19.170006384746,17.1391221009559,-21.1174551044213));
#100975=CARTESIAN_POINT('Ctrl Pts',(-19.1304434962872,17.1314388632321,
-21.1150556719566));
#100976=CARTESIAN_POINT('Ctrl Pts',(-19.1232921207835,17.1300882746966,
-21.1146204235108));
#100977=CARTESIAN_POINT('Ctrl Pts',(-19.1120820261218,17.1280309763835,
-21.1139355616461));
#100978=CARTESIAN_POINT('Ctrl Pts',(-19.1080278880933,17.1272991793239,
-21.113687351279));
#100979=CARTESIAN_POINT('Ctrl Pts',(-19.1004544984534,17.1259549499233,
-21.1132226466908));
#100980=CARTESIAN_POINT('Ctrl Pts',(-19.0969358244336,17.1253395897244,
-21.1130063210192));
#100981=CARTESIAN_POINT('Ctrl Pts',(-19.0889105109887,17.1239570134916,
-21.1125119826549));
#100982=CARTESIAN_POINT('Ctrl Pts',(-19.0844029522625,17.1231954908363,
-21.1122336521205));
#100983=CARTESIAN_POINT('Ctrl Pts',(-19.0726563214473,17.1212500862499,
-21.111506628694));
#100984=CARTESIAN_POINT('Ctrl Pts',(-19.0654135712445,17.120089230196,-21.1110566820063));
#100985=CARTESIAN_POINT('Ctrl Pts',(-19.0185462950184,17.1128270472442,
-21.108134916606));
#100986=CARTESIAN_POINT('Ctrl Pts',(-18.9787639863779,17.1078151658732,
-21.1056078731911));
#100987=CARTESIAN_POINT('Ctrl Pts',(-18.9293667005263,17.1030123453667,
-21.10243141649));
#100988=CARTESIAN_POINT('Ctrl Pts',(-18.9198608688469,17.1021529614027,
-21.101818379856));
#100989=CARTESIAN_POINT('Ctrl Pts',(-18.9031213067476,17.1007536641103,
-21.1007360681414));
#100990=CARTESIAN_POINT('Ctrl Pts',(-18.8958899391321,17.100186588023,-21.1002676096077));
#100991=CARTESIAN_POINT('Ctrl Pts',(-18.7362362311158,17.0884919561016,
-21.0899068464011));
#100992=CARTESIAN_POINT('Ctrl Pts',(-18.5830546826722,17.0938640484914,
-21.0796431322706));
#100993=CARTESIAN_POINT('Ctrl Pts',(-18.3399085143707,17.1289344740535,
-21.0636989433115));
#100994=CARTESIAN_POINT('Ctrl Pts',(-18.248999002911,17.1482147657485,-21.0578086437992));
#100995=CARTESIAN_POINT('Ctrl Pts',(-18.1393450836464,17.1791242524669,
-21.0508127870644));
#100996=CARTESIAN_POINT('Ctrl Pts',(-18.1191382116848,17.1851474499124,
-21.0495279174345));
#100997=CARTESIAN_POINT('Ctrl Pts',(-18.0904788198603,17.1941584763851,
-21.0477111912655));
#100998=CARTESIAN_POINT('Ctrl Pts',(-18.0819505774123,17.1968995072183,
-21.0471712941368));
#100999=CARTESIAN_POINT('Ctrl Pts',(-18.0672481701988,17.2017281244331,
-21.0462416846104));
#101000=CARTESIAN_POINT('Ctrl Pts',(-18.0610658247117,17.2037902277812,
-21.0458511393867));
#101001=CARTESIAN_POINT('Ctrl Pts',(-18.0492329237,17.2077978726255,-21.0451042869256));
#101002=CARTESIAN_POINT('Ctrl Pts',(-18.0435808997982,17.2097388528464,
-21.0447478333971));
#101003=CARTESIAN_POINT('Ctrl Pts',(-18.0288749934262,17.2148587721622,
-21.0438210793781));
#101004=CARTESIAN_POINT('Ctrl Pts',(-18.0198343062371,17.2180754046305,
-21.0432520333695));
#101005=CARTESIAN_POINT('Ctrl Pts',(-17.9889266955431,17.229309510024,-21.0413087397583));
#101006=CARTESIAN_POINT('Ctrl Pts',(-17.9671698833289,17.2376264766844,
-21.0399444668155));
#101007=CARTESIAN_POINT('Ctrl Pts',(-17.7867453367255,17.3100319687421,
-21.0286508791931));
#101008=CARTESIAN_POINT('Ctrl Pts',(-17.6362495753156,17.392780616265,-21.0194297122358));
#101009=CARTESIAN_POINT('Ctrl Pts',(-17.4241895045278,17.5454041718357,
-21.0052229945768));
#101010=CARTESIAN_POINT('Ctrl Pts',(-17.3544763511468,17.6026701463593,
-21.0002984137781));
#101011=CARTESIAN_POINT('Ctrl Pts',(-17.2604233414268,17.6905556007389,
-20.9929548669999));
#101012=CARTESIAN_POINT('Ctrl Pts',(-17.2329445862863,17.7176776763696,
-20.990713732154));
#101013=CARTESIAN_POINT('Ctrl Pts',(-17.2009529130676,17.7510295810089,
-20.9879643250547));
#101014=CARTESIAN_POINT('Ctrl Pts',(-17.1957109990217,17.7565537340423,
-20.9875091393365));
#101015=CARTESIAN_POINT('Ctrl Pts',(-17.1876303376171,17.7651620296073,
-20.9867999110871));
#101016=CARTESIAN_POINT('Ctrl Pts',(-17.1847706914004,17.7682265881143,
-20.9865474425624));
#101017=CARTESIAN_POINT('Ctrl Pts',(-17.1794973579274,17.7739115447412,
-20.9860790832809));
#101018=CARTESIAN_POINT('Ctrl Pts',(-17.1770811768264,17.776529550696,-20.985863387877));
#101019=CARTESIAN_POINT('Ctrl Pts',(-17.171650206002,17.7824440588812,-20.9853760793965));
#101020=CARTESIAN_POINT('Ctrl Pts',(-17.168639253863,17.7857439916569,-20.9851041836218));
#101021=CARTESIAN_POINT('Ctrl Pts',(-17.1598305600817,17.7954596965133,
-20.9843037090298));
#101022=CARTESIAN_POINT('Ctrl Pts',(-17.1540617387684,17.8019014011743,
-20.9837730352611));
#101023=CARTESIAN_POINT('Ctrl Pts',(-17.1140886154277,17.847091111986,-20.9800517939001));
#101024=CARTESIAN_POINT('Ctrl Pts',(-17.0812767165212,17.8870418646467,
-20.9767700694316));
#101025=CARTESIAN_POINT('Ctrl Pts',(-17.0366049255505,17.9456838931232,
-20.9720108784507));
#101026=CARTESIAN_POINT('Ctrl Pts',(-17.0235224619813,17.9634257801954,
-20.9705781363113));
#101027=CARTESIAN_POINT('Ctrl Pts',(-16.9840416998996,18.0187565066996,
-20.9661386995925));
#101028=CARTESIAN_POINT('Ctrl Pts',(-16.9585880704776,18.0570022160794,
-20.9631104032372));
#101029=CARTESIAN_POINT('Ctrl Pts',(-16.8768044981679,18.1890055004216,
-20.952852536024));
#101030=CARTESIAN_POINT('Ctrl Pts',(-16.8264950267668,18.286296732229,-20.9456215479727));
#101031=CARTESIAN_POINT('Ctrl Pts',(-16.7624918150616,18.4377746827603,
-20.935051674093));
#101032=CARTESIAN_POINT('Ctrl Pts',(-16.743043719579,18.4893242944996,-20.9315643799399));
#101033=CARTESIAN_POINT('Ctrl Pts',(-16.7147841334681,18.5741075002619,
-20.9260094669004));
#101034=CARTESIAN_POINT('Ctrl Pts',(-16.7047328255545,18.6068975892386,
-20.9239034475204));
#101035=CARTESIAN_POINT('Ctrl Pts',(-16.692567015497,18.6503243895863,-20.9211678961681));
#101036=CARTESIAN_POINT('Ctrl Pts',(-16.6897316565199,18.6607521313475,
-20.9205150390416));
#101037=CARTESIAN_POINT('Ctrl Pts',(-16.6852176288022,18.677870219475,-20.9194497533633));
#101038=CARTESIAN_POINT('Ctrl Pts',(-16.6834916184812,18.6845477737855,
-20.9190357959774));
#101039=CARTESIAN_POINT('Ctrl Pts',(-16.6802131744755,18.697492107773,-20.9182363927813));
#101040=CARTESIAN_POINT('Ctrl Pts',(-16.6786567166939,18.7037577804726,
-20.9178508207361));
#101041=CARTESIAN_POINT('Ctrl Pts',(-16.6751283426088,18.7182445126901,
-20.916962478573));
#101042=CARTESIAN_POINT('Ctrl Pts',(-16.6731769522369,18.7264704953727,
-20.916460374614));
#101043=CARTESIAN_POINT('Ctrl Pts',(-16.6680598872477,18.7486314794224,
-20.9151138004726));
#101044=CARTESIAN_POINT('Ctrl Pts',(-16.6649859067855,18.7625873604674,
-20.9142722722917));
#101045=CARTESIAN_POINT('Ctrl Pts',(-16.6380608291297,18.8910033987868,
-20.9065856922688));
#101046=CARTESIAN_POINT('Ctrl Pts',(-16.6235871694191,19.0072310393739,
-20.9000578439795));
#101047=CARTESIAN_POINT('Ctrl Pts',(-16.6120973750738,19.2868148923392,
-20.8847399161451));
#101048=CARTESIAN_POINT('Ctrl Pts',(-16.6242137074027,19.4497645786932,
-20.8761331037338));
#101049=CARTESIAN_POINT('Ctrl Pts',(-16.6609680124453,19.6414320748346,
-20.8649250547471));
#101050=CARTESIAN_POINT('Ctrl Pts',(-16.6677798589054,19.6730253932406,
-20.8630398995738));
#101051=CARTESIAN_POINT('Ctrl Pts',(-16.676995934903,19.7114752634247,-20.8606856482955));
#101052=CARTESIAN_POINT('Ctrl Pts',(-16.6787161391372,19.7184933112644,
-20.8602534748482));
#101053=CARTESIAN_POINT('Ctrl Pts',(-16.6814701905088,19.729485528465,-20.8595725042855));
#101054=CARTESIAN_POINT('Ctrl Pts',(-16.6824797484422,19.7334658064096,
-20.8593250865489));
#101055=CARTESIAN_POINT('Ctrl Pts',(-16.6843891937364,19.7409031078772,
-20.8588611648892));
#101056=CARTESIAN_POINT('Ctrl Pts',(-16.6852862528948,19.7443607996941,
-20.8586448251508));
#101057=CARTESIAN_POINT('Ctrl Pts',(-16.6873549100026,19.7522521645731,
-20.8581495888958));
#101058=CARTESIAN_POINT('Ctrl Pts',(-16.6885321618239,19.7566842971341,
-20.857870368922));
#101059=CARTESIAN_POINT('Ctrl Pts',(-16.6921981460778,19.7703074816635,
-20.8570088909108));
#101060=CARTESIAN_POINT('Ctrl Pts',(-16.6947344562219,19.7794854473959,
-20.8564239797095));
#101061=CARTESIAN_POINT('Ctrl Pts',(-16.7185343451424,19.8633992576212,
-20.8510365618186));
#101062=CARTESIAN_POINT('Ctrl Pts',(-16.7438334688544,19.936920850802,-20.8460297370155));
#101063=CARTESIAN_POINT('Ctrl Pts',(-16.7885257179879,20.0467579655339,
-20.8382685750025));
#101064=CARTESIAN_POINT('Ctrl Pts',(-16.8050335551802,20.0841837645915,
-20.835571509564));
#101065=CARTESIAN_POINT('Ctrl Pts',(-16.8696061976661,20.2197976882591,
-20.8256494079995));
#101066=CARTESIAN_POINT('Ctrl Pts',(-16.9241744076404,20.3147082127857,
-20.8184221012403));
#101067=CARTESIAN_POINT('Ctrl Pts',(-17.0168586001139,20.4504114142015,
-20.8078599064588));
#101068=CARTESIAN_POINT('Ctrl Pts',(-17.0496456073477,20.4946145597812,
-20.804376610865));
#101069=CARTESIAN_POINT('Ctrl Pts',(-17.1055890392046,20.5641964861083,
-20.7988272183826));
#101070=CARTESIAN_POINT('Ctrl Pts',(-17.1277042687642,20.5903756655214,
-20.7967228268436));
#101071=CARTESIAN_POINT('Ctrl Pts',(-17.1576168855612,20.6240895262534,
-20.7939889661635));
#101072=CARTESIAN_POINT('Ctrl Pts',(-17.1648493283023,20.632116430481,-20.793336214705));
#101073=CARTESIAN_POINT('Ctrl Pts',(-17.1767991111987,20.6451764067874,
-20.7922710048987));
#101074=CARTESIAN_POINT('Ctrl Pts',(-17.1814800943103,20.6502423416708,
-20.7918570189909));
#101075=CARTESIAN_POINT('Ctrl Pts',(-17.1905913556545,20.6600067138341,
-20.7910574934934));
#101076=CARTESIAN_POINT('Ctrl Pts',(-17.1950185320719,20.6647079290479,
-20.7906718279997));
#101077=CARTESIAN_POINT('Ctrl Pts',(-17.2052936953164,20.6755195689603,
-20.7897831737492));
#101078=CARTESIAN_POINT('Ctrl Pts',(-17.211156953004,20.6816153784147,-20.789280851952));
#101079=CARTESIAN_POINT('Ctrl Pts',(-17.2270311388425,20.6979224365489,
-20.7879334761326));
#101080=CARTESIAN_POINT('Ctrl Pts',(-17.2371093648017,20.708067774687,-20.7870913683861));
#101081=CARTESIAN_POINT('Ctrl Pts',(-17.3310032720836,20.8006907364185,
-20.7793648727674));
#101082=CARTESIAN_POINT('Ctrl Pts',(-17.4214563952892,20.876157973595,-20.7728015699113));
#101083=CARTESIAN_POINT('Ctrl Pts',(-17.6516586437018,21.037747046402,-20.7574080994725));
#101084=CARTESIAN_POINT('Ctrl Pts',(-17.7960287030646,21.115905529318,-20.7487612801579));
#101085=CARTESIAN_POINT('Ctrl Pts',(-17.9767197820359,21.1881637888426,
-20.7375685778981));
#101086=CARTESIAN_POINT('Ctrl Pts',(-18.0057508617983,21.1990399746008,
-20.7357583833923));
#101087=CARTESIAN_POINT('Ctrl Pts',(-18.0417424942445,21.2116297611677,
-20.7334875428134));
#101088=CARTESIAN_POINT('Ctrl Pts',(-18.048488264599,21.2139512108072,-20.7330607897004));
#101089=CARTESIAN_POINT('Ctrl Pts',(-18.0591164770944,21.2175487613245,
-20.7323864470807));
#101090=CARTESIAN_POINT('Ctrl Pts',(-18.0629911723919,21.2188478163658,
-20.7321401922051));
#101091=CARTESIAN_POINT('Ctrl Pts',(-18.0702630954118,21.2212624473527,
-20.7316772137967));
#101092=CARTESIAN_POINT('Ctrl Pts',(-18.0736593962089,21.2223806382822,
-20.7314606469632));
#101093=CARTESIAN_POINT('Ctrl Pts',(-18.0814483292277,21.2249231964012,
-20.7309632227257));
#101094=CARTESIAN_POINT('Ctrl Pts',(-18.0858427868814,21.2263417948775,
-20.7306820311186));
#101095=CARTESIAN_POINT('Ctrl Pts',(-18.0994689231671,21.2306913445902,
-20.7298085049893));
#101096=CARTESIAN_POINT('Ctrl Pts',(-18.1087159491924,21.2335732774126,
-20.7292134107893));
#101097=CARTESIAN_POINT('Ctrl Pts',(-18.2199126560322,21.2673934772227,
-20.7220325508895));
#101098=CARTESIAN_POINT('Ctrl Pts',(-18.3240264479709,21.2906529106698,
-20.7150668263269));
#101099=CARTESIAN_POINT('Ctrl Pts',(-18.5377423054188,21.321722761019,-20.7008203925458));
#101100=CARTESIAN_POINT('Ctrl Pts',(-18.6471161595362,21.3290466606485,
-20.6935600582885));
#101101=CARTESIAN_POINT('Ctrl Pts',(-18.8191820635797,21.3272121252008,
-20.6824360458578));
#101102=CARTESIAN_POINT('Ctrl Pts',(-18.8817380677183,21.3237669956584,
-20.6784511134523));
#101103=CARTESIAN_POINT('Ctrl Pts',(-18.9688268937871,21.3150829634757,
-20.6729960955378));
#101104=CARTESIAN_POINT('Ctrl Pts',(-18.9935548418232,21.3121758977807,
-20.6714575322988));
#101105=CARTESIAN_POINT('Ctrl Pts',(-19.0367601328771,21.3063221945307,
-20.6687868757669));
#101106=CARTESIAN_POINT('Ctrl Pts',(-19.0552600187143,21.3035656100988,
-20.667649001354));
#101107=CARTESIAN_POINT('Ctrl Pts',(-19.082145839258,21.299194512327,-20.6660031598973));
#101108=CARTESIAN_POINT('Ctrl Pts',(-19.0905619898507,21.2977739210157,
-20.6654890767733));
#101109=CARTESIAN_POINT('Ctrl Pts',(-19.1053191349361,21.2951911270328,
-20.664589567943));
#101110=CARTESIAN_POINT('Ctrl Pts',(-19.1116637979455,21.2940507941765,
-20.6642034528007));
#101111=CARTESIAN_POINT('Ctrl Pts',(-19.1239855933328,21.2917780380252,
-20.6634547557497));
#101112=CARTESIAN_POINT('Ctrl Pts',(-19.1299632416492,21.2906487970295,
-20.6630920767236));
#101113=CARTESIAN_POINT('Ctrl Pts',(-19.1442608459029,21.2878839479357,
-20.662225845325));
#101114=CARTESIAN_POINT('Ctrl Pts',(-19.1525760472977,21.2862240820405,
-20.6617230701115));
#101115=CARTESIAN_POINT('Ctrl Pts',(-19.1826608302047,21.2800304297158,
-20.6599074744352));
#101116=CARTESIAN_POINT('Ctrl Pts',(-19.204369094039,21.27520358256,-20.6586040075469));
#101117=CARTESIAN_POINT('Ctrl Pts',(-19.4052504162273,21.2272038315851,
-20.646593406177));
#101118=CARTESIAN_POINT('Ctrl Pts',(-19.5781382614978,21.161151721059,-20.6367288607255));
#101119=CARTESIAN_POINT('Ctrl Pts',(-19.8115607126271,21.035037415791,-20.6222695482745));
#101120=CARTESIAN_POINT('Ctrl Pts',(-19.8805486379102,20.9924807747384,
-20.6178178032159));
#101121=CARTESIAN_POINT('Ctrl Pts',(-19.9766416479195,20.9253061314895,
-20.6111129213783));
#101122=CARTESIAN_POINT('Ctrl Pts',(-20.0058193888798,20.9037725378276,
-20.6090041897175));
#101123=CARTESIAN_POINT('Ctrl Pts',(-20.0403302052841,20.8769070639192,
-20.6064015535575));
#101124=CARTESIAN_POINT('Ctrl Pts',(-20.0462081228253,20.872281068771,-20.6059543652548));
#101125=CARTESIAN_POINT('Ctrl Pts',(-20.0553184316746,20.8650326256605,
-20.6052549397604));
#101126=CARTESIAN_POINT('Ctrl Pts',(-20.0585678799266,20.8624315775757,
-20.6050042074991));
#101127=CARTESIAN_POINT('Ctrl Pts',(-20.0645866185924,20.857584635999,-20.6045373987949));
#101128=CARTESIAN_POINT('Ctrl Pts',(-20.0673579134824,20.8553413231554,
-20.604321507035));
#101129=CARTESIAN_POINT('Ctrl Pts',(-20.0736189686333,20.8502468777262,
-20.6038315983027));
#101130=CARTESIAN_POINT('Ctrl Pts',(-20.0771052823971,20.8473916116828,
-20.6035572852201));
#101131=CARTESIAN_POINT('Ctrl Pts',(-20.0873944146572,20.8389098545557,
-20.6027432679808));
#101132=CARTESIAN_POINT('Ctrl Pts',(-20.0941710862548,20.8332519983257,
-20.6022013638953));
#101133=CARTESIAN_POINT('Ctrl Pts',(-20.143789056171,20.7912964047527,-20.5981921760178));
#101134=CARTESIAN_POINT('Ctrl Pts',(-20.1852027882272,20.7533524859523,
-20.5946174055716));
#101135=CARTESIAN_POINT('Ctrl Pts',(-20.2694056946639,20.6698082744742,
-20.5869377264677));
#101136=CARTESIAN_POINT('Ctrl Pts',(-20.3117845642145,20.6238649911955,
-20.5828224214743));
#101137=CARTESIAN_POINT('Ctrl Pts',(-20.4227518412588,20.4923359103383,
-20.5714554666818));
#101138=CARTESIAN_POINT('Ctrl Pts',(-20.4868272471835,20.4031847999859,
-20.5642058558508));
#101139=CARTESIAN_POINT('Ctrl Pts',(-20.5724488758391,20.2621240945041,
-20.5535968573673));
#101140=CARTESIAN_POINT('Ctrl Pts',(-20.5993182072117,20.2136689133617,
-20.5500892113808));
#101141=CARTESIAN_POINT('Ctrl Pts',(-20.6397608240933,20.1334695794462,
-20.5445056329858));
#101142=CARTESIAN_POINT('Ctrl Pts',(-20.6545119640231,20.1023520395552,
-20.542390810797));
#101143=CARTESIAN_POINT('Ctrl Pts',(-20.6728942756066,20.0609971313829,
-20.5396456255145));
#101144=CARTESIAN_POINT('Ctrl Pts',(-20.6772145010782,20.0510735354429,
-20.5389917354065));
#101145=CARTESIAN_POINT('Ctrl Pts',(-20.6841645607711,20.0347686637089,
-20.5379251655332));
#101146=CARTESIAN_POINT('Ctrl Pts',(-20.6868395890268,20.0284069773867,
-20.5375109503167));
#101147=CARTESIAN_POINT('Ctrl Pts',(-20.6919565565327,20.0160694343696,
-20.5367113258279));
#101148=CARTESIAN_POINT('Ctrl Pts',(-20.69440236109,20.010095273095,-20.5363257888581));
#101149=CARTESIAN_POINT('Ctrl Pts',(-20.6999852443612,19.9962785263683,
-20.535437921984));
#101150=CARTESIAN_POINT('Ctrl Pts',(-20.7031028023643,19.9884281329464,
-20.534936255541));
#101151=CARTESIAN_POINT('Ctrl Pts',(-20.7113578704912,19.9672726128737,
-20.533591727848));
#101152=CARTESIAN_POINT('Ctrl Pts',(-20.7164081045861,19.953933735049,-20.5327517937283));
#101153=CARTESIAN_POINT('Ctrl Pts',(-20.7714922868465,19.8038811168905,
-20.5233872789514));
#101154=CARTESIAN_POINT('Ctrl Pts',(-20.807433641414,19.6624018986933,-20.5153747723651));
#101155=CARTESIAN_POINT('Ctrl Pts',(-20.8435716232148,19.416112685353,-20.5018390757858));
#101156=CARTESIAN_POINT('Ctrl Pts',(-20.8510665768693,19.3129337983554,
-20.4962758775061));
#101157=CARTESIAN_POINT('Ctrl Pts',(-20.8509605930263,19.1495719709784,
-20.4871374802086));
#101158=CARTESIAN_POINT('Ctrl Pts',(-20.8483662200053,19.089551891809,-20.4837077513012));
#101159=CARTESIAN_POINT('Ctrl Pts',(-20.8424571664132,19.0207954149847,
-20.4796145097686));
#101160=CARTESIAN_POINT('Ctrl Pts',(-20.841632618508,19.0118665127582,-20.4790797464361));
#101161=CARTESIAN_POINT('Ctrl Pts',(-20.8403055954211,18.9984292733184,
-20.4782697850337));
#101162=CARTESIAN_POINT('Ctrl Pts',(-20.8398453013716,18.9939167418798,
-20.4779968993075));
#101163=CARTESIAN_POINT('Ctrl Pts',(-20.8389970519398,18.985857509629,-20.4775079023638));
#101164=CARTESIAN_POINT('Ctrl Pts',(-20.8386146300039,18.982310278849,-20.4772921050407));
#101165=CARTESIAN_POINT('Ctrl Pts',(-20.8377689780624,18.9746480716415,
-20.4768247302818));
#101166=CARTESIAN_POINT('Ctrl Pts',(-20.8373026477863,18.9705335403155,
-20.4765729858425));
#101167=CARTESIAN_POINT('Ctrl Pts',(-20.8359714187925,18.959088018593,-20.4758706109915));
#101168=CARTESIAN_POINT('Ctrl Pts',(-20.8350802526843,18.9517602270393,
-20.4754185410009));
#101169=CARTESIAN_POINT('Ctrl Pts',(-20.8297855227008,18.9100449594236,
-20.4728319942608));
#101170=CARTESIAN_POINT('Ctrl Pts',(-20.8245763661117,18.8757672010279,
-20.4706561904851));
#101171=CARTESIAN_POINT('Ctrl Pts',(-20.805407187068,18.7675849999349,-20.4636610960151));
#101172=CARTESIAN_POINT('Ctrl Pts',(-20.7883503387104,18.6942914438053,
-20.4587324781192));
#101173=CARTESIAN_POINT('Ctrl Pts',(-20.7540340414928,18.5758063603463,
-20.4505956795289));
#101174=CARTESIAN_POINT('Ctrl Pts',(-20.7390724281762,18.5300554743709,
-20.4474104160584));
#101175=CARTESIAN_POINT('Ctrl Pts',(-20.7225807433525,18.4848900722567,
-20.4442393203449));
#101176=CARTESIAN_POINT('Origin',(-18.734,19.211,0.));
#101177=CARTESIAN_POINT('',(-20.7225806138715,18.48488971765,-19.6425236773711));
#101178=CARTESIAN_POINT('',(-20.7227695130846,18.4848207703082,-19.8664843328284));
#101179=CARTESIAN_POINT('',(-20.7225806137986,18.4848897174502,0.));
#101180=CARTESIAN_POINT('',(-20.8479202214574,19.2118282579775,-19.9109991817851));
#101181=CARTESIAN_POINT('Ctrl Pts',(-20.7227695130846,18.4848207703082,
-19.8664843328284));
#101182=CARTESIAN_POINT('Ctrl Pts',(-20.804884879996,18.7170154428126,-19.8813041288781));
#101183=CARTESIAN_POINT('Ctrl Pts',(-20.8469525585721,18.9645595409249,
-19.8961239249278));
#101184=CARTESIAN_POINT('Ctrl Pts',(-20.8478239854299,19.2118314138294,
-19.9109437209775));
#101185=CARTESIAN_POINT('Ctrl Pts',(-20.8509998750784,19.2117272674116,
-19.9127739856851));
#101186=CARTESIAN_POINT('Ctrl Pts',(-20.8509329967896,19.4064030179171,
-19.9239833448391));
#101187=CARTESIAN_POINT('Ctrl Pts',(-20.8240164289188,19.6001371512442,
-19.9342646615468));
#101188=CARTESIAN_POINT('Ctrl Pts',(-20.7539266223477,19.8478012358022,
-19.9484105777364));
#101189=CARTESIAN_POINT('Ctrl Pts',(-20.7341848393677,19.9073324161759,
-19.9519023179064));
#101190=CARTESIAN_POINT('Ctrl Pts',(-20.7008063068113,19.9947844856038,
-19.9572865274355));
#101191=CARTESIAN_POINT('Ctrl Pts',(-20.6891489403589,20.0234269582284,
-19.9590922948951));
#101192=CARTESIAN_POINT('Ctrl Pts',(-20.6740381883075,20.0583438718382,
-19.9613581802236));
#101193=CARTESIAN_POINT('Ctrl Pts',(-20.6711741838903,20.064871177176,-19.9617845754105));
#101194=CARTESIAN_POINT('Ctrl Pts',(-20.6666170558022,20.0751163138349,
-19.9624584640114));
#101195=CARTESIAN_POINT('Ctrl Pts',(-20.6649460109109,20.0788439897307,
-19.9627046254899));
#101196=CARTESIAN_POINT('Ctrl Pts',(-20.6617920753916,20.0858254111333,
-19.9631675124283));
#101197=CARTESIAN_POINT('Ctrl Pts',(-20.6603117270743,20.0890802442623,
-19.9633840817028));
#101198=CARTESIAN_POINT('Ctrl Pts',(-20.6568999796044,20.0965314836647,
-19.9638816154836));
#101199=CARTESIAN_POINT('Ctrl Pts',(-20.6549630916597,20.1007253169778,
-19.9641629148743));
#101200=CARTESIAN_POINT('Ctrl Pts',(-20.6489187115762,20.113701126155,-19.9650371214703));
#101201=CARTESIAN_POINT('Ctrl Pts',(-20.6447646744777,20.1224611048584,
-19.9656327945442));
#101202=CARTESIAN_POINT('Ctrl Pts',(-20.5974958425972,20.2203976442717,
-19.9723516834412));
#101203=CARTESIAN_POINT('Ctrl Pts',(-20.5482381121763,20.3064614442048,
-19.978804301781));
#101204=CARTESIAN_POINT('Ctrl Pts',(-20.3994520607462,20.5286955145451,
-19.9964221181772));
#101205=CARTESIAN_POINT('Ctrl Pts',(-20.2893760933458,20.656985506077,-20.0076101401363));
#101206=CARTESIAN_POINT('Ctrl Pts',(-20.142381265471,20.7918586839756,-20.0201370322126));
#101207=CARTESIAN_POINT('Ctrl Pts',(-20.1190566221779,20.8123339058851,
-20.0220657955069));
#101208=CARTESIAN_POINT('Ctrl Pts',(-20.083694192387,20.8420253874502,-20.0249044937089));
#101209=CARTESIAN_POINT('Ctrl Pts',(-20.0719947948906,20.8516365151964,
-20.0258302504258));
#101210=CARTESIAN_POINT('Ctrl Pts',(-20.0530931164119,20.8668276842146,
-20.0273048426957));
#101211=CARTESIAN_POINT('Ctrl Pts',(-20.0459563402534,20.8724880483815,
-20.0278568908671));
#101212=CARTESIAN_POINT('Ctrl Pts',(-20.032275018599,20.8831959448073,-20.0289062961756));
#101213=CARTESIAN_POINT('Ctrl Pts',(-20.0257370300029,20.888251546457,-20.0294039696052));
#101214=CARTESIAN_POINT('Ctrl Pts',(-20.0142093374607,20.8970581291556,
-20.0302748583175));
#101215=CARTESIAN_POINT('Ctrl Pts',(-20.0092323688278,20.9008255440729,
-20.0306487201506));
#101216=CARTESIAN_POINT('Ctrl Pts',(-19.9993768526463,20.9082175337247,
-20.0313848825214));
#101217=CARTESIAN_POINT('Ctrl Pts',(-19.9944992178411,20.9118432199949,
-20.031747224437));
#101218=CARTESIAN_POINT('Ctrl Pts',(-19.9827969500719,20.9204638635275,
-20.0326118280847));
#101219=CARTESIAN_POINT('Ctrl Pts',(-19.9759578325285,20.9254390536238,
-20.0331133193308));
#101220=CARTESIAN_POINT('Ctrl Pts',(-19.9511436683167,20.9432639806312,
-20.0349193587283));
#101221=CARTESIAN_POINT('Ctrl Pts',(-19.9329971415061,20.9558733813039,
-20.0362146834485));
#101222=CARTESIAN_POINT('Ctrl Pts',(-19.7605626419638,21.0717316823665,
-20.0482971339985));
#101223=CARTESIAN_POINT('Ctrl Pts',(-19.5935258037612,21.1545469264989,
-20.058226996901));
#101224=CARTESIAN_POINT('Ctrl Pts',(-19.3420019683425,21.2403940052829,
-20.0727154285207));
#101225=CARTESIAN_POINT('Ctrl Pts',(-19.2647854177626,21.2619439918426,
-20.0771209800648));
#101226=CARTESIAN_POINT('Ctrl Pts',(-19.1513519633396,21.2867658503118,
-20.0837630738697));
#101227=CARTESIAN_POINT('Ctrl Pts',(-19.1159749302518,21.2935660447937,
-20.0858583070635));
#101228=CARTESIAN_POINT('Ctrl Pts',(-19.073079047516,21.30068182661,-20.0884459728523));
#101229=CARTESIAN_POINT('Ctrl Pts',(-19.0657076913315,21.3018645916638,
-20.0888923157214));
#101230=CARTESIAN_POINT('Ctrl Pts',(-19.0542202447418,21.3036455251472,
-20.0895907064303));
#101231=CARTESIAN_POINT('Ctrl Pts',(-19.0501083029054,21.3042706082139,
-20.0898412565919));
#101232=CARTESIAN_POINT('Ctrl Pts',(-19.0424675729422,21.3054090986372,
-20.0903079091407));
#101233=CARTESIAN_POINT('Ctrl Pts',(-19.0389393200879,21.3059257090573,
-20.0905238279943));
#101234=CARTESIAN_POINT('Ctrl Pts',(-19.030944958559,21.3070756280897,-20.0910140347372));
#101235=CARTESIAN_POINT('Ctrl Pts',(-19.0264781434004,21.3077035751025,
-20.0912886202271));
#101236=CARTESIAN_POINT('Ctrl Pts',(-19.0149391402234,21.3092881429337,
-20.0919996560863));
#101237=CARTESIAN_POINT('Ctrl Pts',(-19.0078641268994,21.3102232773034,
-20.0924372735682));
#101238=CARTESIAN_POINT('Ctrl Pts',(-18.9643736385953,21.3157479995676,
-20.0951369196823));
#101239=CARTESIAN_POINT('Ctrl Pts',(-18.927850962396,21.3194253804304,-20.0974452298616));
#101240=CARTESIAN_POINT('Ctrl Pts',(-18.7213619389661,21.334806177892,-20.110659789649));
#101241=CARTESIAN_POINT('Ctrl Pts',(-18.5505653489567,21.3269081264315,
-20.1221547076964));
#101242=CARTESIAN_POINT('Ctrl Pts',(-18.2884045167855,21.2827745397975,
-20.1394321265249));
#101243=CARTESIAN_POINT('Ctrl Pts',(-18.1954218306955,21.2605713935224,
-20.1454985875449));
#101244=CARTESIAN_POINT('Ctrl Pts',(-18.0838108543755,21.2257955611563,
-20.1526795157099));
#101245=CARTESIAN_POINT('Ctrl Pts',(-18.0634741698727,21.2191190806999,
-20.1539841059781));
#101246=CARTESIAN_POINT('Ctrl Pts',(-18.0347231103209,21.2091946959523,
-20.1558235730162));
#101247=CARTESIAN_POINT('Ctrl Pts',(-18.0262233551174,21.2061998487007,
-20.1563667679624));
#101248=CARTESIAN_POINT('Ctrl Pts',(-18.0116010459551,21.2009425493188,
-20.1573002560387));
#101249=CARTESIAN_POINT('Ctrl Pts',(-18.0054694057941,21.1987059071154,
-20.1576914007262));
#101250=CARTESIAN_POINT('Ctrl Pts',(-17.9937544296498,21.194371137569,-20.1584381760808));
#101251=CARTESIAN_POINT('Ctrl Pts',(-17.9881694343077,21.1922777044536,
-20.1587939589084));
#101252=CARTESIAN_POINT('Ctrl Pts',(-17.9736814654561,21.1867772128867,
-20.1597163216899));
#101253=CARTESIAN_POINT('Ctrl Pts',(-17.9647924607477,21.1833335506472,
-20.1602816708529));
#101254=CARTESIAN_POINT('Ctrl Pts',(-17.9346222919521,21.1714104300775,
-20.1621988566334));
#101255=CARTESIAN_POINT('Ctrl Pts',(-17.9134551616601,21.1626454603826,
-20.1635410827725));
#101256=CARTESIAN_POINT('Ctrl Pts',(-17.7304080204605,21.0833439233905,
-20.1751339207498));
#101257=CARTESIAN_POINT('Ctrl Pts',(-17.5778023356978,20.9931566251877,
-20.1846226481057));
#101258=CARTESIAN_POINT('Ctrl Pts',(-17.3699603892135,20.8322717347333,
-20.1989262911642));
#101259=CARTESIAN_POINT('Ctrl Pts',(-17.3050599679199,20.7753702029045,
-20.2036497927853));
#101260=CARTESIAN_POINT('Ctrl Pts',(-17.2170884180828,20.6881879279199,
-20.2107225725073));
#101261=CARTESIAN_POINT('Ctrl Pts',(-17.1910740434533,20.6609944899403,
-20.2129086417915));
#101262=CARTESIAN_POINT('Ctrl Pts',(-17.1607209933252,20.6275236777881,
-20.2155970395049));
#101263=CARTESIAN_POINT('Ctrl Pts',(-17.1556721850282,20.621895980275,-20.2160489851472));
#101264=CARTESIAN_POINT('Ctrl Pts',(-17.1478791669026,20.6131152499366,
-20.2167542503612));
#101265=CARTESIAN_POINT('Ctrl Pts',(-17.1451139090301,20.6099808649583,
-20.2170060241879));
#101266=CARTESIAN_POINT('Ctrl Pts',(-17.1400080879926,20.604158815895,-20.2174737723779));
#101267=CARTESIAN_POINT('Ctrl Pts',(-17.1376650223745,20.6014734231465,
-20.2176895557201));
#101268=CARTESIAN_POINT('Ctrl Pts',(-17.1323898274841,20.5953966029653,
-20.2181779338014));
#101269=CARTESIAN_POINT('Ctrl Pts',(-17.1294617005161,20.5920017898766,
-20.2184508166558));
#101270=CARTESIAN_POINT('Ctrl Pts',(-17.1208698812539,20.5819763902115,
-20.2192567625331));
#101271=CARTESIAN_POINT('Ctrl Pts',(-17.1152364292426,20.5753201744836,
-20.2197919623718));
#101272=CARTESIAN_POINT('Ctrl Pts',(-17.0754280443729,20.5276908507112,
-20.2236211945399));
#101273=CARTESIAN_POINT('Ctrl Pts',(-17.0427745988218,20.4854768864669,
-20.2270123268198));
#101274=CARTESIAN_POINT('Ctrl Pts',(-17.0014698657048,20.4276926691785,
-20.2316028871494));
#101275=CARTESIAN_POINT('Ctrl Pts',(-16.9913672212685,20.4131783109953,
-20.2327518680578));
#101276=CARTESIAN_POINT('Ctrl Pts',(-16.9542828102629,20.358449712802,-20.2370647154527));
#101277=CARTESIAN_POINT('Ctrl Pts',(-16.928502063074,20.3174407268073,-20.2402571474152));
#101278=CARTESIAN_POINT('Ctrl Pts',(-16.8491453205084,20.1810393442284,
-20.2506814069089));
#101279=CARTESIAN_POINT('Ctrl Pts',(-16.8015457833797,20.0823653990544,
-20.2579141799284));
#101280=CARTESIAN_POINT('Ctrl Pts',(-16.7417565160167,19.9291163151288,
-20.2684877832564));
#101281=CARTESIAN_POINT('Ctrl Pts',(-16.7237398566363,19.8770181068162,
-20.2719769928328));
#101282=CARTESIAN_POINT('Ctrl Pts',(-16.6978380967518,19.791439864176,-20.2775346565794));
#101283=CARTESIAN_POINT('Ctrl Pts',(-16.6886997911586,19.7583691662929,
-20.2796415520352));
#101284=CARTESIAN_POINT('Ctrl Pts',(-16.6777441127393,19.714604554195,-20.2823781060041));
#101285=CARTESIAN_POINT('Ctrl Pts',(-16.6751997194972,19.7040996174073,
-20.2830311069466));
#101286=CARTESIAN_POINT('Ctrl Pts',(-16.6711634531294,19.6868591832121,
-20.2840965978255));
#101287=CARTESIAN_POINT('Ctrl Pts',(-16.6696238752665,19.6801351604117,
-20.284510617228));
#101288=CARTESIAN_POINT('Ctrl Pts',(-16.6667068937383,19.6671029497557,
-20.285310120112));
#101289=CARTESIAN_POINT('Ctrl Pts',(-16.6653254325331,19.6607957573325,
-20.2856957299459));
#101290=CARTESIAN_POINT('Ctrl Pts',(-16.6622017498403,19.6462154501031,
-20.2865841308635));
#101291=CARTESIAN_POINT('Ctrl Pts',(-16.6604801817904,19.6379379861622,
-20.2870862559163));
#101292=CARTESIAN_POINT('Ctrl Pts',(-16.6559824261701,19.6156432341906,
-20.2884328251107));
#101293=CARTESIAN_POINT('Ctrl Pts',(-16.6532984651169,19.6016076314751,
-20.2892743280243));
#101294=CARTESIAN_POINT('Ctrl Pts',(-16.6299799881091,19.4725978897857,
-20.2969546135082));
#101295=CARTESIAN_POINT('Ctrl Pts',(-16.6187508688479,19.35612077854,-20.3034768593072));
#101296=CARTESIAN_POINT('Ctrl Pts',(-16.6150144513764,19.0766239483158,
-20.3187792468033));
#101297=CARTESIAN_POINT('Ctrl Pts',(-16.6315987518409,18.9142613277445,
-20.32737647937));
#101298=CARTESIAN_POINT('Ctrl Pts',(-16.6736109104469,18.7236124388203,
-20.3385851003764));
#101299=CARTESIAN_POINT('Ctrl Pts',(-16.6813527832375,18.6919730488902,
-20.340484669114));
#101300=CARTESIAN_POINT('Ctrl Pts',(-16.6917044350884,18.6535322451149,
-20.3428549836005));
#101301=CARTESIAN_POINT('Ctrl Pts',(-16.6936238539226,18.6465474765195,
-20.3432882160116));
#101302=CARTESIAN_POINT('Ctrl Pts',(-16.6966885873772,18.6356148205229,
-20.3439705047836));
#101303=CARTESIAN_POINT('Ctrl Pts',(-16.6978096390778,18.6316601082338,
-20.3442181733064));
#101304=CARTESIAN_POINT('Ctrl Pts',(-16.6999263046096,18.6242752271231,
-20.3446823147868));
#101305=CARTESIAN_POINT('Ctrl Pts',(-16.7009190838304,18.620844304409,-20.3448986220296));
#101306=CARTESIAN_POINT('Ctrl Pts',(-16.7032047245649,18.6130196275873,
-20.3453934677246));
#101307=CARTESIAN_POINT('Ctrl Pts',(-16.7045031605318,18.6086275618869,
-20.3456723275607));
#101308=CARTESIAN_POINT('Ctrl Pts',(-16.7085366015657,18.5951451990489,
-20.3465316486347));
#101309=CARTESIAN_POINT('Ctrl Pts',(-16.7113184618293,18.5860692024863,
-20.3471147443886));
#101310=CARTESIAN_POINT('Ctrl Pts',(-16.7367817781939,18.504944909698,-20.3523662003622));
#101311=CARTESIAN_POINT('Ctrl Pts',(-16.7632408399181,18.4341472256021,
-20.3572277648161));
#101312=CARTESIAN_POINT('Ctrl Pts',(-16.8475388062047,18.2407998437208,
-20.3710207776939));
#101313=CARTESIAN_POINT('Ctrl Pts',(-16.9134444274173,18.1221449755099,
-20.380071654904));
#101314=CARTESIAN_POINT('Ctrl Pts',(-17.0412232627869,17.9365264809378,
-20.3946755832312));
#101315=CARTESIAN_POINT('Ctrl Pts',(-17.0968871011714,17.8657711017126,
-20.400374317523));
#101316=CARTESIAN_POINT('Ctrl Pts',(-17.1707190562842,17.7833195617048,
-20.4071681362679));
#101317=CARTESIAN_POINT('Ctrl Pts',(-17.1847745268805,17.7680796195588,
-20.4084311588121));
#101318=CARTESIAN_POINT('Ctrl Pts',(-17.2051791613217,17.7465973921756,
-20.4102226229612));
#101319=CARTESIAN_POINT('Ctrl Pts',(-17.2113470127651,17.7401852465992,
-20.4107588038578));
#101320=CARTESIAN_POINT('Ctrl Pts',(-17.2220949648835,17.7291516629236,
-20.4116840330176));
#101321=CARTESIAN_POINT('Ctrl Pts',(-17.2266562504447,17.7245121421788,
-20.4120738932576));
#101322=CARTESIAN_POINT('Ctrl Pts',(-17.2354572831088,17.7156423188519,
-20.4128208258324));
#101323=CARTESIAN_POINT('Ctrl Pts',(-17.2396937293779,17.7114088425072,
-20.4131780377929));
#101324=CARTESIAN_POINT('Ctrl Pts',(-17.2508157881043,17.7003885130447,
-20.4141098133903));
#101325=CARTESIAN_POINT('Ctrl Pts',(-17.2577300776067,17.6936307002295,
-20.4146830950959));
#101326=CARTESIAN_POINT('Ctrl Pts',(-17.2817710489933,17.6704536774689,
-20.4166561462286));
#101327=CARTESIAN_POINT('Ctrl Pts',(-17.2991276785304,17.6542747879271,
-20.4180455186176));
#101328=CARTESIAN_POINT('Ctrl Pts',(-17.4372220490245,17.5298231529634,
-20.4288399098562));
#101329=CARTESIAN_POINT('Ctrl Pts',(-17.5697669392347,17.435455854964,-20.4376192523952));
#101330=CARTESIAN_POINT('Ctrl Pts',(-17.826002806886,17.2941698767093,-20.4535153747511));
#101331=CARTESIAN_POINT('Ctrl Pts',(-17.9457644034907,17.241895789985,-20.4606076528614));
#101332=CARTESIAN_POINT('Ctrl Pts',(-18.0808431626167,17.1972431688575,
-20.4690033218645));
#101333=CARTESIAN_POINT('Ctrl Pts',(-18.092165579344,17.1936058909993,-20.4697100607116));
#101334=CARTESIAN_POINT('Ctrl Pts',(-18.1083099118619,17.188569256165,-20.470722839672));
#101335=CARTESIAN_POINT('Ctrl Pts',(-18.1131073251388,17.1870912853774,
-20.4710244270176));
#101336=CARTESIAN_POINT('Ctrl Pts',(-18.1213857891815,17.1845730882951,
-20.4715460102468));
#101337=CARTESIAN_POINT('Ctrl Pts',(-18.1248643808242,17.1835247234353,
-20.4717655314615));
#101338=CARTESIAN_POINT('Ctrl Pts',(-18.1316159712677,17.1815088986904,
-20.4721923107604));
#101339=CARTESIAN_POINT('Ctrl Pts',(-18.134888617637,17.1805403969773,-20.4723995005998));
#101340=CARTESIAN_POINT('Ctrl Pts',(-18.143727874773,17.1779477519314,-20.4729599469651));
#101341=CARTESIAN_POINT('Ctrl Pts',(-18.1492987920689,17.1763385734176,
-20.4733140610665));
#101342=CARTESIAN_POINT('Ctrl Pts',(-18.1700194199307,17.17044547435,-20.4746342979861));
#101343=CARTESIAN_POINT('Ctrl Pts',(-18.1852097317425,17.166307828859,-20.4756083763569));
#101344=CARTESIAN_POINT('Ctrl Pts',(-18.3278725961528,17.1291525194958,
-20.4848055002339));
#101345=CARTESIAN_POINT('Ctrl Pts',(-18.4581078740452,17.1079294301442,
-20.4935470591748));
#101346=CARTESIAN_POINT('Ctrl Pts',(-18.7483666258248,17.0880649382775,
-20.512765243392));
#101347=CARTESIAN_POINT('Ctrl Pts',(-18.9080248088637,17.0951566177402,
-20.523134715843));
#101348=CARTESIAN_POINT('Ctrl Pts',(-19.0864174187945,17.1234311203351,
-20.5342281069483));
#101349=CARTESIAN_POINT('Ctrl Pts',(-19.1073848159156,17.1270792492146,
-20.5355251447755));
#101350=CARTESIAN_POINT('Ctrl Pts',(-19.1371282788457,17.132717671934,-20.5373559214712));
#101351=CARTESIAN_POINT('Ctrl Pts',(-19.1459516440063,17.1344486061607,
-20.5378978712834));
#101352=CARTESIAN_POINT('Ctrl Pts',(-19.161156975732,17.1375322593507,-20.5388299066604));
#101353=CARTESIAN_POINT('Ctrl Pts',(-19.1675441579279,17.1388583499106,
-20.5392208366072));
#101354=CARTESIAN_POINT('Ctrl Pts',(-19.1797638916366,17.1414543536714,
-20.5399676695837));
#101355=CARTESIAN_POINT('Ctrl Pts',(-19.1855973918155,17.1427194517779,
-20.5403237225325));
#101356=CARTESIAN_POINT('Ctrl Pts',(-19.200756728963,17.1460742163823,-20.5412477970872));
#101357=CARTESIAN_POINT('Ctrl Pts',(-19.210073971578,17.1482024059497,-20.5418145788388));
#101358=CARTESIAN_POINT('Ctrl Pts',(-19.2418174041233,17.155679583403,-20.5437418189165));
#101359=CARTESIAN_POINT('Ctrl Pts',(-19.2641709741738,17.1613318975078,
-20.5450925279138));
#101360=CARTESIAN_POINT('Ctrl Pts',(-19.4549969360399,17.2129148995966,
-20.5565784041027));
#101361=CARTESIAN_POINT('Ctrl Pts',(-19.6172789241533,17.2791600141646,
-20.5659713132975));
#101362=CARTESIAN_POINT('Ctrl Pts',(-19.8460072152757,17.4074466969931,
-20.5802385721217));
#101363=CARTESIAN_POINT('Ctrl Pts',(-19.9196794697496,17.455002753997,-20.5850329924141));
#101364=CARTESIAN_POINT('Ctrl Pts',(-20.0207558647494,17.5295153697323,
-20.5922013954482));
#101365=CARTESIAN_POINT('Ctrl Pts',(-20.0507099894184,17.5528668276205,
-20.594407091961));
#101366=CARTESIAN_POINT('Ctrl Pts',(-20.0858687975861,17.5818292848284,
-20.597117248846));
#101367=CARTESIAN_POINT('Ctrl Pts',(-20.0916937737515,17.5866804261975,
-20.5975703739912));
#101368=CARTESIAN_POINT('Ctrl Pts',(-20.1006932904131,17.5942576092888,
-20.5982770887487));
#101369=CARTESIAN_POINT('Ctrl Pts',(-20.1038860824254,17.5969620114556,
-20.5985291224611));
#101370=CARTESIAN_POINT('Ctrl Pts',(-20.1097830253455,17.6019870215249,
-20.5989970938741));
#101371=CARTESIAN_POINT('Ctrl Pts',(-20.1124893426084,17.6043049979944,
-20.5992128389032));
#101372=CARTESIAN_POINT('Ctrl Pts',(-20.1185827491747,17.6095507641986,
-20.5997008031928));
#101373=CARTESIAN_POINT('Ctrl Pts',(-20.1219663903594,17.6124824547283,
-20.5999733084864));
#101374=CARTESIAN_POINT('Ctrl Pts',(-20.1318927161188,17.6211382053024,
-20.600777214251));
#101375=CARTESIAN_POINT('Ctrl Pts',(-20.1384093794245,17.6268917773528,
-20.601310736214));
#101376=CARTESIAN_POINT('Ctrl Pts',(-20.1842711531029,17.667888625123,-20.6051052317313));
#101377=CARTESIAN_POINT('Ctrl Pts',(-20.2223172484895,17.7045505680284,
-20.6084614050717));
#101378=CARTESIAN_POINT('Ctrl Pts',(-20.2724917961696,17.7566571257431,
-20.6131348661714));
#101379=CARTESIAN_POINT('Ctrl Pts',(-20.2858389487213,17.7709076254727,
-20.6144037567851));
#101380=CARTESIAN_POINT('Ctrl Pts',(-20.3975967056274,17.8935872679086,
-20.6252363275479));
#101381=CARTESIAN_POINT('Ctrl Pts',(-20.4847193340846,18.0117847032248,
-20.635041563272));
#101382=CARTESIAN_POINT('Ctrl Pts',(-20.5902290418307,18.1912387775492,
-20.6484906099546));
#101383=CARTESIAN_POINT('Ctrl Pts',(-20.6191743051358,18.2457963052028,
-20.652416720791));
#101384=CARTESIAN_POINT('Ctrl Pts',(-20.6616864794049,18.3351579187673,
-20.6585827206034));
#101385=CARTESIAN_POINT('Ctrl Pts',(-20.6767885690955,18.3691880460116,
-20.6608723820402));
#101386=CARTESIAN_POINT('Ctrl Pts',(-20.6952311498234,18.4138894314091,
-20.6638069544908));
#101387=CARTESIAN_POINT('Ctrl Pts',(-20.6993949387512,18.4242118304521,
-20.6644796438639));
#101388=CARTESIAN_POINT('Ctrl Pts',(-20.7060329030986,18.4410494907003,
-20.6655690059949));
#101389=CARTESIAN_POINT('Ctrl Pts',(-20.7085566166865,18.4475448755945,
-20.6659873429946));
#101390=CARTESIAN_POINT('Ctrl Pts',(-20.7133473834865,18.4600577369324,
-20.6667896316462));
#101391=CARTESIAN_POINT('Ctrl Pts',(-20.7156191778918,18.4660733041461,
-20.6671737389019));
#101392=CARTESIAN_POINT('Ctrl Pts',(-20.7194496212452,18.476357603124,-20.6678277322614));
#101393=CARTESIAN_POINT('Ctrl Pts',(-20.7210219845465,18.4806211373333,
-20.6680980731543));
#101394=CARTESIAN_POINT('Ctrl Pts',(-20.7225806137969,18.4848897174457,
-20.6683679590049));
#101395=CARTESIAN_POINT('',(-20.8509992561167,19.2127747116643,-19.6896815252242));
#101396=CARTESIAN_POINT('Ctrl Pts',(-20.7225807433526,18.4848900722567,
-20.4442393203449));
#101397=CARTESIAN_POINT('Ctrl Pts',(-20.6728906059831,18.3488048232718,
-20.4346846760922));
#101398=CARTESIAN_POINT('Ctrl Pts',(-20.6093080638511,18.2180329568345,
-20.4252946696087));
#101399=CARTESIAN_POINT('Ctrl Pts',(-20.5215596808033,18.076641000874,-20.4150700053436));
#101400=CARTESIAN_POINT('Ctrl Pts',(-20.5100907656587,18.0587666924442,
-20.4137751521916));
#101401=CARTESIAN_POINT('Ctrl Pts',(-20.4937578192524,18.0341352659228,
-20.4119870263363));
#101402=CARTESIAN_POINT('Ctrl Pts',(-20.489120264994,18.0272301561407,-20.4114853253551));
#101403=CARTESIAN_POINT('Ctrl Pts',(-20.4810444660834,18.0153574414848,
-20.410621905054));
#101404=CARTESIAN_POINT('Ctrl Pts',(-20.4776254578743,18.010376929243,-20.4102594642419));
#101405=CARTESIAN_POINT('Ctrl Pts',(-20.4705005833394,18.0000926601601,
-20.4095105249595));
#101406=CARTESIAN_POINT('Ctrl Pts',(-20.4667916236948,17.9947911150203,
-20.4091241495084));
#101407=CARTESIAN_POINT('Ctrl Pts',(-20.4580472077302,17.9824131472918,
-20.4082213013032));
#101408=CARTESIAN_POINT('Ctrl Pts',(-20.4529923702198,17.9753505093745,
-20.4077055785196));
#101409=CARTESIAN_POINT('Ctrl Pts',(-20.4364321499066,17.9525108047212,
-20.4060357450383));
#101410=CARTESIAN_POINT('Ctrl Pts',(-20.4247517091076,17.9368614770944,
-20.4048884148582));
#101411=CARTESIAN_POINT('Ctrl Pts',(-20.3638544321887,17.8575843122734,
-20.3990559677338));
#101412=CARTESIAN_POINT('Ctrl Pts',(-20.3112538502044,17.796633773947,-20.3945074746445));
#101413=CARTESIAN_POINT('Ctrl Pts',(-20.138483026706,17.6180975957617,-20.3807326283317));
#101414=CARTESIAN_POINT('Ctrl Pts',(-20.0077165243318,17.5117208941659,
-20.3718907614783));
#101415=CARTESIAN_POINT('Ctrl Pts',(-19.8645530330822,17.4211561819165,
-20.3623782531059));
#101416=CARTESIAN_POINT('Ctrl Pts',(-19.8633411537126,17.420391273265,-20.3622977373751));
#101417=CARTESIAN_POINT('Ctrl Pts',(-19.81655501399,17.3909273954177,-20.3591895853458));
#101418=CARTESIAN_POINT('Ctrl Pts',(-19.7699069101227,17.3639792984401,
-20.3561002921224));
#101419=CARTESIAN_POINT('Ctrl Pts',(-19.7145584441951,17.3347616067901,
-20.3523863368298));
#101420=CARTESIAN_POINT('Ctrl Pts',(-19.7068050888467,17.33072990669,-20.3518649966277));
#101421=CARTESIAN_POINT('Ctrl Pts',(-19.6950331765953,17.3247008801767,
-20.3510714814948));
#101422=CARTESIAN_POINT('Ctrl Pts',(-19.6910327562121,17.3226680803822,
-20.3508014819472));
#101423=CARTESIAN_POINT('Ctrl Pts',(-19.6838432653658,17.3190434795445,
-20.3503155779541));
#101424=CARTESIAN_POINT('Ctrl Pts',(-19.6806566133226,17.3174470009492,
-20.3500999709661));
#101425=CARTESIAN_POINT('Ctrl Pts',(-19.6737268225542,17.313997115266,-20.3496305813145));
#101426=CARTESIAN_POINT('Ctrl Pts',(-19.6699822753743,17.3121467604877,
-20.3493766185275));
#101427=CARTESIAN_POINT('Ctrl Pts',(-19.6594568561791,17.3069843599479,
-20.3486619023854));
#101428=CARTESIAN_POINT('Ctrl Pts',(-19.6526637936787,17.303697512072,-20.3481996277763));
#101429=CARTESIAN_POINT('Ctrl Pts',(-19.6121138579633,17.2843441626581,
-20.3454348739854));
#101430=CARTESIAN_POINT('Ctrl Pts',(-19.5779559774992,17.2691388890306,
-20.3430842637068));
#101431=CARTESIAN_POINT('Ctrl Pts',(-19.4646091700166,17.2222383027167,
-20.3352555019467));
#101432=CARTESIAN_POINT('Ctrl Pts',(-19.3839086960102,17.1944237767704,
-20.3296395655382));
#101433=CARTESIAN_POINT('Ctrl Pts',(-19.1303563755561,17.1238379271948,
-20.3122523962994));
#101434=CARTESIAN_POINT('Ctrl Pts',(-18.9535875700027,17.0979099373504,
-20.3005610254208));
#101435=CARTESIAN_POINT('Ctrl Pts',(-18.752839403414,17.0939610479623,-20.2882045288104));
#101436=CARTESIAN_POINT('Ctrl Pts',(-18.7300372273483,17.0938809178972,
-20.2868128276617));
#101437=CARTESIAN_POINT('Ctrl Pts',(-18.6977234993785,17.0942894515593,
-20.2848566749309));
#101438=CARTESIAN_POINT('Ctrl Pts',(-18.6882103146583,17.0944738745489,
-20.2842827535119));
#101439=CARTESIAN_POINT('Ctrl Pts',(-18.6727394882684,17.0948781498583,
-20.283352537761));
#101440=CARTESIAN_POINT('Ctrl Pts',(-18.6667810406777,17.0950590396748,
-20.2829950275873));
#101441=CARTESIAN_POINT('Ctrl Pts',(-18.6542977717837,17.0954907966553,
-20.2822475745448));
#101442=CARTESIAN_POINT('Ctrl Pts',(-18.6477731783199,17.0957466886174,
-20.2818577931372));
#101443=CARTESIAN_POINT('Ctrl Pts',(-18.632231273506,17.0964282663284,-20.2809313804777));
#101444=CARTESIAN_POINT('Ctrl Pts',(-18.6232152485678,17.0968814524183,
-20.2803956165752));
#101445=CARTESIAN_POINT('Ctrl Pts',(-18.5927418222677,17.0986086635144,
-20.2785901794381));
#101446=CARTESIAN_POINT('Ctrl Pts',(-18.5713005723079,17.1001518345607,
-20.2773289409156));
#101447=CARTESIAN_POINT('Ctrl Pts',(-18.3710912248426,17.1176301312793,
-20.2656276868687));
#101448=CARTESIAN_POINT('Ctrl Pts',(-18.1950096865446,17.155909585088,-20.2559846656249));
#101449=CARTESIAN_POINT('Ctrl Pts',(-17.9123224784601,17.2562496983917,
-20.239659495714));
#101450=CARTESIAN_POINT('Ctrl Pts',(-17.8024525421218,17.3061604911142,
-20.2330499538334));
#101451=CARTESIAN_POINT('Ctrl Pts',(-17.6891592405312,17.3697811165665,
-20.2253492287921));
#101452=CARTESIAN_POINT('Ctrl Pts',(-17.6809102776687,17.3744866680367,
-20.2247831552277));
#101453=CARTESIAN_POINT('Ctrl Pts',(-17.668729829774,17.3815439474008,-20.223938864268));
#101454=CARTESIAN_POINT('Ctrl Pts',(-17.6647737376536,17.3838532672582,
-20.2236633191161));
#101455=CARTESIAN_POINT('Ctrl Pts',(-17.6577463291092,17.3879860686191,
-20.223171430173));
#101456=CARTESIAN_POINT('Ctrl Pts',(-17.6546721017577,17.389804500895,-20.2229554153578));
#101457=CARTESIAN_POINT('Ctrl Pts',(-17.6480701593711,17.393732195175,-20.2224897131493));
#101458=CARTESIAN_POINT('Ctrl Pts',(-17.6445440323422,17.3958439221123,
-20.2222398701498));
#101459=CARTESIAN_POINT('Ctrl Pts',(-17.6348222554596,17.4017046324115,
-20.2215480153092));
#101460=CARTESIAN_POINT('Ctrl Pts',(-17.6286397260923,17.4054751171345,
-20.2211046318912));
#101461=CARTESIAN_POINT('Ctrl Pts',(-17.5947844377301,17.4263612041883,
-20.2186584702281));
#101462=CARTESIAN_POINT('Ctrl Pts',(-17.5674913724603,17.4440803409526,
-20.2166193474724));
#101463=CARTESIAN_POINT('Ctrl Pts',(-17.4062323924254,17.5541372896315,
-20.2042133326344));
#101464=CARTESIAN_POINT('Ctrl Pts',(-17.2828701653958,17.6610377443148,
-20.1932565596486));
#101465=CARTESIAN_POINT('Ctrl Pts',(-17.0940658716516,17.8671437397052,
-20.1749990462804));
#101466=CARTESIAN_POINT('Ctrl Pts',(-17.0224173953814,17.9596701525316,
-20.1675583081085));
#101467=CARTESIAN_POINT('Ctrl Pts',(-16.9509757827139,18.0696333521042,
-20.1595513474906));
#101468=CARTESIAN_POINT('Ctrl Pts',(-16.9433122896736,18.081694583312,-20.1586833737028));
#101469=CARTESIAN_POINT('Ctrl Pts',(-16.9313098110433,18.1010141617528,
-20.1573090685292));
#101470=CARTESIAN_POINT('Ctrl Pts',(-16.9268912795455,18.1082223459977,
-20.156799809085));
#101471=CARTESIAN_POINT('Ctrl Pts',(-16.9191746656097,18.1209817915745,
-20.155904432912));
#101472=CARTESIAN_POINT('Ctrl Pts',(-16.9158585990382,18.126521998109,-20.1555176600582));
#101473=CARTESIAN_POINT('Ctrl Pts',(-16.9090523342738,18.1380123018482,
-20.1547195928986));
#101474=CARTESIAN_POINT('Ctrl Pts',(-16.9055657637645,18.143964467078,-20.1543084339737));
#101475=CARTESIAN_POINT('Ctrl Pts',(-16.896690896535,18.1592865956576,-20.1532557261412));
#101476=CARTESIAN_POINT('Ctrl Pts',(-16.8913451116359,18.1686810490569,
-20.1526157185331));
#101477=CARTESIAN_POINT('Ctrl Pts',(-16.8693339928606,18.208061058517,-20.1499550578646));
#101478=CARTESIAN_POINT('Ctrl Pts',(-16.853326246324,18.2384095068536,-20.1479579335101));
#101479=CARTESIAN_POINT('Ctrl Pts',(-16.813545968641,18.3184856500672,-20.1428138659717));
#101480=CARTESIAN_POINT('Ctrl Pts',(-16.7909645796331,18.3687770176533,
-20.1397063117002));
#101481=CARTESIAN_POINT('Ctrl Pts',(-16.729508374182,18.5213196846395,-20.1305619110663));
#101482=CARTESIAN_POINT('Ctrl Pts',(-16.6965650566323,18.625760433208,-20.1246737943342));
#101483=CARTESIAN_POINT('Ctrl Pts',(-16.6614983193697,18.7768154286109,
-20.116231033899));
#101484=CARTESIAN_POINT('Ctrl Pts',(-16.6526050361312,18.8216746533904,
-20.1137310759661));
#101485=CARTESIAN_POINT('Ctrl Pts',(-16.6414626797021,18.8892907854021,
-20.109931173351));
#101486=CARTESIAN_POINT('Ctrl Pts',(-16.6381180741534,18.9118542887672,
-20.1086578632305));
#101487=CARTESIAN_POINT('Ctrl Pts',(-16.6349974222111,18.9355397495938,
-20.1073117924615));
#101488=CARTESIAN_POINT('Ctrl Pts',(-16.6348568850456,18.9366127662384,
-20.1072507914662));
#101489=CARTESIAN_POINT('Ctrl Pts',(-16.6322374465911,18.9567322622386,
-20.1061066103224));
#101490=CARTESIAN_POINT('Ctrl Pts',(-16.6300171109765,18.9758109798522,
-20.1050151058199));
#101491=CARTESIAN_POINT('Ctrl Pts',(-16.6247209031575,19.0274277145969,
-20.1020383098619));
#101492=CARTESIAN_POINT('Ctrl Pts',(-16.6221385626885,19.0600096082949,
-20.1001338376914));
#101493=CARTESIAN_POINT('Ctrl Pts',(-16.6199272709424,19.0994978606305,
-20.0977810017928));
#101494=CARTESIAN_POINT('Ctrl Pts',(-16.6195764447247,19.1063613035157,
-20.0973704250738));
#101495=CARTESIAN_POINT('Ctrl Pts',(-16.6190544600331,19.1176512677001,
-20.0966921914135));
#101496=CARTESIAN_POINT('Ctrl Pts',(-16.6188637624841,19.122076894036,-20.096425604087));
#101497=CARTESIAN_POINT('Ctrl Pts',(-16.6185448279198,19.1300611628517,
-20.0959432995976));
#101498=CARTESIAN_POINT('Ctrl Pts',(-16.6184116783697,19.1336195536188,
-20.0957278604086));
#101499=CARTESIAN_POINT('Ctrl Pts',(-16.6181402572395,19.141398419221,-20.0952558208679));
#101500=CARTESIAN_POINT('Ctrl Pts',(-16.618005636687,19.1456189263562,-20.0949990237828));
#101501=CARTESIAN_POINT('Ctrl Pts',(-16.6176594987087,19.1575951432613,
-20.0942684353934));
#101502=CARTESIAN_POINT('Ctrl Pts',(-16.6174779917045,19.1653515579983,
-20.0937930147968));
#101503=CARTESIAN_POINT('Ctrl Pts',(-16.6166002516263,19.2143832865097,
-20.090774172285));
#101504=CARTESIAN_POINT('Ctrl Pts',(-16.6170688673251,19.2556676444565,
-20.0881719902205));
#101505=CARTESIAN_POINT('Ctrl Pts',(-16.6263056167701,19.4830965564417,
-20.0735979883229));
#101506=CARTESIAN_POINT('Ctrl Pts',(-16.6584150814937,19.667474680233,-20.0609880542896));
#101507=CARTESIAN_POINT('Ctrl Pts',(-16.7265097397931,19.8843092161046,
-20.0463553693014));
#101508=CARTESIAN_POINT('Ctrl Pts',(-16.7398954494216,19.9229759886991,
-20.0437495378147));
#101509=CARTESIAN_POINT('Ctrl Pts',(-16.7714206331086,20.0061601274996,
-20.038155973527));
#101510=CARTESIAN_POINT('Ctrl Pts',(-16.7899728257612,20.0504976674327,
-20.0351826552735));
#101511=CARTESIAN_POINT('Ctrl Pts',(-16.8152563240624,20.1055777254093,
-20.0314966012245));
#101512=CARTESIAN_POINT('Ctrl Pts',(-16.8205950248732,20.1169404023194,
-20.0307365803096));
#101513=CARTESIAN_POINT('Ctrl Pts',(-16.829222354364,20.1348859510944,-20.0295367007417));
#101514=CARTESIAN_POINT('Ctrl Pts',(-16.8324447082229,20.1415001904288,
-20.0290945558979));
#101515=CARTESIAN_POINT('Ctrl Pts',(-16.8385177147121,20.1538024090151,
-20.0282723197112));
#101516=CARTESIAN_POINT('Ctrl Pts',(-16.8413596455273,20.159494578937,-20.0278919298622));
#101517=CARTESIAN_POINT('Ctrl Pts',(-16.8477345680061,20.1721203225221,
-20.0270482709653));
#101518=CARTESIAN_POINT('Ctrl Pts',(-16.8512802274971,20.1790474239422,
-20.0265854523787));
#101519=CARTESIAN_POINT('Ctrl Pts',(-16.8617121017617,20.1991539030193,
-20.0252421315433));
#101520=CARTESIAN_POINT('Ctrl Pts',(-16.868699165901,20.2122806425408,-20.0243651931879));
#101521=CARTESIAN_POINT('Ctrl Pts',(-16.9263126056649,20.3178238053714,
-20.0173123880134));
#101522=CARTESIAN_POINT('Ctrl Pts',(-16.9836392822435,20.4064221959172,
-20.0113903529587));
#101523=CARTESIAN_POINT('Ctrl Pts',(-17.1506102904383,20.6265458347475,
-19.9961927724823));
#101524=CARTESIAN_POINT('Ctrl Pts',(-17.2699801424405,20.7496769061546,
-19.9872040129537));
#101525=CARTESIAN_POINT('Ctrl Pts',(-17.4310700848671,20.8799462121164,
-19.9753651326896));
#101526=CARTESIAN_POINT('Ctrl Pts',(-17.4598889608157,20.9020495346235,
-19.9732549007287));
#101527=CARTESIAN_POINT('Ctrl Pts',(-17.4950130511549,20.9275811739013,
-19.9706731292046));
#101528=CARTESIAN_POINT('Ctrl Pts',(-17.5007870632448,20.9317339815871,
-19.9702484037449));
#101529=CARTESIAN_POINT('Ctrl Pts',(-17.5102509758777,20.9384685543212,
-19.9695515550325));
#101530=CARTESIAN_POINT('Ctrl Pts',(-17.5139284352826,20.9410678184152,
-19.969280604102));
#101531=CARTESIAN_POINT('Ctrl Pts',(-17.5205321909445,20.9457038906499,
-19.9687936860607));
#101532=CARTESIAN_POINT('Ctrl Pts',(-17.5234553626189,20.9477450568451,
-19.968578021834));
#101533=CARTESIAN_POINT('Ctrl Pts',(-17.5298043194842,20.952154532896,-19.9681093209745));
#101534=CARTESIAN_POINT('Ctrl Pts',(-17.5332318947952,20.9545200891387,
-19.9678561086374));
#101535=CARTESIAN_POINT('Ctrl Pts',(-17.542843949844,20.9611121036239,-19.9671455732856));
#101536=CARTESIAN_POINT('Ctrl Pts',(-17.5490438430358,20.9653158248424,
-19.9666867569045));
#101537=CARTESIAN_POINT('Ctrl Pts',(-17.5855322703882,20.9897744472999,
-19.9639840988715));
#101538=CARTESIAN_POINT('Ctrl Pts',(-17.6163154316405,21.0092762570028,
-19.9616945576796));
#101539=CARTESIAN_POINT('Ctrl Pts',(-17.7176718529215,21.0698799307747,
-19.9541639183685));
#101540=CARTESIAN_POINT('Ctrl Pts',(-17.790121126065,21.1076940730335,-19.9487955231222));
#101541=CARTESIAN_POINT('Ctrl Pts',(-18.0316576092181,21.2164893821606,
-19.9313020627634));
#101542=CARTESIAN_POINT('Ctrl Pts',(-18.2078510505483,21.2697536045674,
-19.9192368835383));
#101543=CARTESIAN_POINT('Ctrl Pts',(-18.4107597067682,21.3032962078264,
-19.9065862044123));
#101544=CARTESIAN_POINT('Ctrl Pts',(-18.4328493528678,21.3065896678846,
-19.9052235065917));
#101545=CARTESIAN_POINT('Ctrl Pts',(-18.4634073217987,21.310652529906,-19.903357762854));
#101546=CARTESIAN_POINT('Ctrl Pts',(-18.4718337372479,21.3117213041717,
-19.9028453020299));
#101547=CARTESIAN_POINT('Ctrl Pts',(-18.4863097608782,21.313468929447,-19.9019683343136));
#101548=CARTESIAN_POINT('Ctrl Pts',(-18.4923562347127,21.3141724479337,
-19.9016030528011));
#101549=CARTESIAN_POINT('Ctrl Pts',(-18.5048099557765,21.3155670462917,
-19.9008527586787));
#101550=CARTESIAN_POINT('Ctrl Pts',(-18.5112174982534,21.3162549696037,
-19.9004678492857));
#101551=CARTESIAN_POINT('Ctrl Pts',(-18.5261056533957,21.3177846514556,
-19.8995760599226));
#101552=CARTESIAN_POINT('Ctrl Pts',(-18.5345884445009,21.3186044841792,
-19.8990698751179));
#101553=CARTESIAN_POINT('Ctrl Pts',(-18.561633245491,21.3210535290192,-19.897462037221));
#101554=CARTESIAN_POINT('Ctrl Pts',(-18.5802122374725,21.3224889415647,
-19.8963664720597));
#101555=CARTESIAN_POINT('Ctrl Pts',(-18.7564804645901,21.3337684677006,
-19.8860513128699));
#101556=CARTESIAN_POINT('Ctrl Pts',(-18.9147901479484,21.3261771440115,
-19.8774371923853));
#101557=CARTESIAN_POINT('Ctrl Pts',(-19.133304647157,21.2909647471643,-19.8654175769343));
#101558=CARTESIAN_POINT('Ctrl Pts',(-19.1953264881964,21.2780933740107,
-19.8619838223684));
#101559=CARTESIAN_POINT('Ctrl Pts',(-19.2922208170295,21.2534064072117,
-19.8564699346951));
#101560=CARTESIAN_POINT('Ctrl Pts',(-19.3275224580092,21.2434284233966,
-19.8544287090835));
#101561=CARTESIAN_POINT('Ctrl Pts',(-19.4078776284072,21.2184440457469,
-19.8496720799651));
#101562=CARTESIAN_POINT('Ctrl Pts',(-19.4527190446368,21.2028295227764,
-19.8469364951043));
#101563=CARTESIAN_POINT('Ctrl Pts',(-19.5041874679935,21.1829431372245,
-19.8436603913552));
#101564=CARTESIAN_POINT('Ctrl Pts',(-19.5113656418058,21.1801244569969,
-19.8432003460221));
#101565=CARTESIAN_POINT('Ctrl Pts',(-19.5228321684879,21.1755493844044,
-19.8424601887408));
#101566=CARTESIAN_POINT('Ctrl Pts',(-19.5271305091645,21.1738179916393,
-19.8421815413537));
#101567=CARTESIAN_POINT('Ctrl Pts',(-19.5347454477853,21.1707215595706,
-19.8416857135591));
#101568=CARTESIAN_POINT('Ctrl Pts',(-19.5380643013971,21.1693621887294,
-19.8414688771737));
#101569=CARTESIAN_POINT('Ctrl Pts',(-19.545105165204,21.1664574022672,-19.8410072758713));
#101570=CARTESIAN_POINT('Ctrl Pts',(-19.5488261634816,21.1649098146488,
-19.8407623856657));
#101571=CARTESIAN_POINT('Ctrl Pts',(-19.5587594185208,21.1607451994584,
-19.8401061763205));
#101572=CARTESIAN_POINT('Ctrl Pts',(-19.5649635720808,21.158109134152,-19.8396937277843));
#101573=CARTESIAN_POINT('Ctrl Pts',(-19.5953243714915,21.1450376858571,
-19.8376630109399));
#101574=CARTESIAN_POINT('Ctrl Pts',(-19.6192964325269,21.1341826544191,
-19.8360211750285));
#101575=CARTESIAN_POINT('Ctrl Pts',(-19.6875994671247,21.1017060739613,
-19.831244645076));
#101576=CARTESIAN_POINT('Ctrl Pts',(-19.7313838060925,21.0789792025445,
-19.8280615524495));
#101577=CARTESIAN_POINT('Ctrl Pts',(-19.8622003523279,21.005166116682,-19.818257712721));
#101578=CARTESIAN_POINT('Ctrl Pts',(-19.9464116339282,20.9493688012213,
-19.8115418948507));
#101579=CARTESIAN_POINT('Ctrl Pts',(-20.0549024968569,20.8657530180286,
-19.8025410873885));
#101580=CARTESIAN_POINT('Ctrl Pts',(-20.0829148471729,20.8429987237112,
-19.8001815409466));
#101581=CARTESIAN_POINT('Ctrl Pts',(-20.1868001578078,20.754110140009,-19.791310017457));
#101582=CARTESIAN_POINT('Ctrl Pts',(-20.2585130730344,20.6833050595772,
-19.7849405203657));
#101583=CARTESIAN_POINT('Ctrl Pts',(-20.3341511245986,20.5971460824146,
-19.7779428091084));
#101584=CARTESIAN_POINT('Ctrl Pts',(-20.3432733702532,20.5865449167058,
-19.7770935587611));
#101585=CARTESIAN_POINT('Ctrl Pts',(-20.3576837179667,20.5694587493837,
-19.7757432252811));
#101586=CARTESIAN_POINT('Ctrl Pts',(-20.3630394689401,20.5630315830412,
-19.7752393709102));
#101587=CARTESIAN_POINT('Ctrl Pts',(-20.3724519313685,20.5515990357681,
-19.7743502625094));
#101588=CARTESIAN_POINT('Ctrl Pts',(-20.3765241311846,20.5466065985188,
-19.7739643812795));
#101589=CARTESIAN_POINT('Ctrl Pts',(-20.3849325598667,20.5362014116365,
-19.7731650172965));
#101590=CARTESIAN_POINT('Ctrl Pts',(-20.3892651129541,20.530785780431,-19.7727516854409));
#101591=CARTESIAN_POINT('Ctrl Pts',(-20.4003867771015,20.5167429403856,
-19.7716868303743));
#101592=CARTESIAN_POINT('Ctrl Pts',(-20.4071355896917,20.5080839690015,
-19.7710369188416));
#101593=CARTESIAN_POINT('Ctrl Pts',(-20.4356099872692,20.470958244399,-19.7682782440148));
#101594=CARTESIAN_POINT('Ctrl Pts',(-20.456679536607,20.4419942173802,-19.7661952793857));
#101595=CARTESIAN_POINT('Ctrl Pts',(-20.5337126838843,20.3302437027319,
-19.7583966171025));
#101596=CARTESIAN_POINT('Ctrl Pts',(-20.5845280728317,20.2440638564465,
-19.7528697247338));
#101597=CARTESIAN_POINT('Ctrl Pts',(-20.6638151472762,20.0848300110632,
-19.7431609957673));
#101598=CARTESIAN_POINT('Ctrl Pts',(-20.6946793403609,20.0131856015894,
-19.7389559408234));
#101599=CARTESIAN_POINT('Ctrl Pts',(-20.7569619472626,19.8433810274421,
-19.7290683047582));
#101600=CARTESIAN_POINT('Ctrl Pts',(-20.7853043460614,19.7443156568392,
-19.723357616558));
#101601=CARTESIAN_POINT('Ctrl Pts',(-20.8083091498158,19.6341127964012,
-19.7166879443766));
#101602=CARTESIAN_POINT('Ctrl Pts',(-20.8102239738572,19.6246144216661,
-19.7161105312899));
#101603=CARTESIAN_POINT('Ctrl Pts',(-20.8129550808653,19.610569896252,-19.7152525410502));
#101604=CARTESIAN_POINT('Ctrl Pts',(-20.8138218293213,19.6060335271828,
-19.7149747635366));
#101605=CARTESIAN_POINT('Ctrl Pts',(-20.8153332624705,19.5979801487786,
-19.7144804213719));
#101606=CARTESIAN_POINT('Ctrl Pts',(-20.8159838885478,19.5944643042486,
-19.7142641983415));
#101607=CARTESIAN_POINT('Ctrl Pts',(-20.8173589116012,19.5869273059115,
-19.7137997822212));
#101608=CARTESIAN_POINT('Ctrl Pts',(-20.8180805645791,19.5829057589892,
-19.7135514426252));
#101609=CARTESIAN_POINT('Ctrl Pts',(-20.819537629611,19.5746485627133,-19.7130404718471));
#101610=CARTESIAN_POINT('Ctrl Pts',(-20.8202717900265,19.5704127141436,
-19.7127777724921));
#101611=CARTESIAN_POINT('Ctrl Pts',(-20.822097106375,19.5596872247049,-19.7121111890396));
#101612=CARTESIAN_POINT('Ctrl Pts',(-20.8231709050189,19.5531947302344,
-19.7117063802511));
#101613=CARTESIAN_POINT('Ctrl Pts',(-20.8419517274706,19.4362562556051,
-19.7043930786085));
#101614=CARTESIAN_POINT('Ctrl Pts',(-20.8509055124935,19.3245986120908,
-19.6970632785419));
#101615=CARTESIAN_POINT('Ctrl Pts',(-20.8509992561167,19.2127747116643,
-19.6896815252242));
#101616=CARTESIAN_POINT('Ctrl Pts',(-20.8509992546756,19.2127764298092,
-19.6896816386429));
#101617=CARTESIAN_POINT('Ctrl Pts',(-20.8510842733145,19.1114583848993,
-19.6829934015258));
#101618=CARTESIAN_POINT('Ctrl Pts',(-20.8438956128816,19.0102558470168,
-19.6762800379215));
#101619=CARTESIAN_POINT('Ctrl Pts',(-20.8169455020383,18.8226665579838,
-19.6640097393302));
#101620=CARTESIAN_POINT('Ctrl Pts',(-20.7989633497378,18.7362425929389,
-19.6584263192726));
#101621=CARTESIAN_POINT('Ctrl Pts',(-20.7702151437283,18.63139866288,-19.6517544981652));
#101622=CARTESIAN_POINT('Ctrl Pts',(-20.7645030418353,18.6116943474891,
-19.6505048401514));
#101623=CARTESIAN_POINT('Ctrl Pts',(-20.755915138356,18.5836032652825,-19.6487288464412));
#101624=CARTESIAN_POINT('Ctrl Pts',(-20.7532718150684,18.5751471632154,
-19.648194953417));
#101625=CARTESIAN_POINT('Ctrl Pts',(-20.748597373308,18.5605165894664,-19.6472724085706));
#101626=CARTESIAN_POINT('Ctrl Pts',(-20.746590773711,18.5543344664484,-19.6468829576124));
#101627=CARTESIAN_POINT('Ctrl Pts',(-20.7426778410948,18.5424655563447,
-19.6461359337708));
#101628=CARTESIAN_POINT('Ctrl Pts',(-20.7407757522879,18.5367774456252,
-19.6457782254421));
#101629=CARTESIAN_POINT('Ctrl Pts',(-20.7357295714009,18.5218976172911,
-19.644843218429));
#101630=CARTESIAN_POINT('Ctrl Pts',(-20.7325463159622,18.5127192551639,
-19.644267219346));
#101631=CARTESIAN_POINT('Ctrl Pts',(-20.72708934705,18.4973280754487,-19.6433024502794));
#101632=CARTESIAN_POINT('Ctrl Pts',(-20.7248495421185,18.4911035763927,
-19.6429125887592));
#101633=CARTESIAN_POINT('Ctrl Pts',(-20.7225806138715,18.48488971765,-19.6425236773711));
#101634=CARTESIAN_POINT('Origin',(-18.734,19.211,0.));
#101635=CARTESIAN_POINT('',(-20.7225806605155,18.4848898453927,-18.8452754875981));
#101636=CARTESIAN_POINT('',(-20.7225806137985,18.4848897174502,-19.0663245303817));
#101637=CARTESIAN_POINT('',(-20.7225806137986,18.4848897174502,0.));
#101638=CARTESIAN_POINT('',(-20.8499620916056,19.2091158126,-19.1109437209775));
#101639=CARTESIAN_POINT('Ctrl Pts',(-20.7225806137985,18.4848897174502,
-19.0663245303817));
#101640=CARTESIAN_POINT('Ctrl Pts',(-20.7389261121638,18.5296547372455,
-19.0692018356968));
#101641=CARTESIAN_POINT('Ctrl Pts',(-20.7537412852729,18.5749225972442,
-19.0720791410119));
#101642=CARTESIAN_POINT('Ctrl Pts',(-20.7670007520343,18.6205790127139,
-19.074956446327));
#101643=CARTESIAN_POINT('Ctrl Pts',(-20.7921933233439,18.7073247712844,
-19.0804232362541));
#101644=CARTESIAN_POINT('Ctrl Pts',(-20.8118478930289,18.7957464915235,
-19.0858900261812));
#101645=CARTESIAN_POINT('Ctrl Pts',(-20.8257819138173,18.8852126076307,
-19.0913568161083));
#101646=CARTESIAN_POINT('Ctrl Pts',(-20.8394880731084,18.9732156942584,
-19.0967342082257));
#101647=CARTESIAN_POINT('Ctrl Pts',(-20.847659220755,19.0622293912709,-19.1021116003431));
#101648=CARTESIAN_POINT('Ctrl Pts',(-20.8501673751634,19.1516313189109,
-19.1074889924605));
#101649=CARTESIAN_POINT('Ctrl Pts',(-20.8507044999982,19.170776868907,-19.1086405686328));
#101650=CARTESIAN_POINT('Ctrl Pts',(-20.8509820862726,19.1899401417876,
-19.1097921448052));
#101651=CARTESIAN_POINT('Ctrl Pts',(-20.8509991606888,19.2091148891276,
-19.1109437209775));
#101652=CARTESIAN_POINT('Ctrl Pts',(-20.8499620916056,19.2091158126,-19.1109437209775));
#101653=CARTESIAN_POINT('Ctrl Pts',(-20.8456332387307,19.7149949859819,
-19.1413398983212));
#101654=CARTESIAN_POINT('Ctrl Pts',(-20.4101935795872,20.9330881089954,
-19.2141280112252));
#101655=CARTESIAN_POINT('Ctrl Pts',(-18.3741968251019,21.6882711019051,
-19.3293080596899));
#101656=CARTESIAN_POINT('Ctrl Pts',(-16.4562524007973,20.2493623486038,
-19.4564838663713));
#101657=CARTESIAN_POINT('Ctrl Pts',(-16.6280000239014,17.8578205442182,
-19.5836596730528));
#101658=CARTESIAN_POINT('Ctrl Pts',(-18.7318719156386,16.7077369880416,
-19.7108354797341));
#101659=CARTESIAN_POINT('Ctrl Pts',(-20.2929105236617,17.5576360808446,
-19.805110366326));
#101660=CARTESIAN_POINT('Ctrl Pts',(-20.670180515561,18.3361167516014,-19.8569933173575));
#101661=CARTESIAN_POINT('Ctrl Pts',(-20.7227695130846,18.4848207703082,
-19.8664843328284));
#101662=CARTESIAN_POINT('Ctrl Pts',(-20.7225806138715,18.48488971765,-19.6425236773711));
#101663=CARTESIAN_POINT('Ctrl Pts',(-20.7166172131094,18.4685578966628,
-19.6415015055718));
#101664=CARTESIAN_POINT('Ctrl Pts',(-20.7104526312527,18.4522995775035,
-19.6404859043171));
#101665=CARTESIAN_POINT('Ctrl Pts',(-20.6487986673468,18.2955482034438,
-19.6307079256196));
#101666=CARTESIAN_POINT('Ctrl Pts',(-20.5786228568079,18.1612956446388,
-19.6224835837011));
#101667=CARTESIAN_POINT('Ctrl Pts',(-20.4575557776264,17.9799307339345,
-19.6106418681866));
#101668=CARTESIAN_POINT('Ctrl Pts',(-20.4177432745747,17.9260159116697,
-19.6070082161425));
#101669=CARTESIAN_POINT('Ctrl Pts',(-20.3413736183221,17.8322507236163,
-19.6003215113211));
#101670=CARTESIAN_POINT('Ctrl Pts',(-20.3057195639882,17.7917409230834,
-19.5972951937388));
#101671=CARTESIAN_POINT('Ctrl Pts',(-20.2493176315369,17.7323919628987,
-19.5925699520392));
#101672=CARTESIAN_POINT('Ctrl Pts',(-20.2296773196887,17.712527965864,-19.5909350015854));
#101673=CARTESIAN_POINT('Ctrl Pts',(-20.2047675548798,17.688312184712,-19.588865181943));
#101674=CARTESIAN_POINT('Ctrl Pts',(-20.1998614349834,17.683588583954,-19.5884576962871));
#101675=CARTESIAN_POINT('Ctrl Pts',(-20.1919761559026,17.6760696375325,
-19.5878028856512));
#101676=CARTESIAN_POINT('Ctrl Pts',(-20.1890115022321,17.673259054155,-19.5875567198869));
#101677=CARTESIAN_POINT('Ctrl Pts',(-20.1834366917092,17.6680045163247,
-19.5870938286371));
#101678=CARTESIAN_POINT('Ctrl Pts',(-20.1808284717707,17.6655585878109,
-19.5868772593599));
#101679=CARTESIAN_POINT('Ctrl Pts',(-20.1748364833881,17.6599679024864,
-19.5863797305478));
#101680=CARTESIAN_POINT('Ctrl Pts',(-20.1714486197794,17.6568276144712,
-19.5860984361602));
#101681=CARTESIAN_POINT('Ctrl Pts',(-20.1609189938946,17.647131344696,-19.5852242629529));
#101682=CARTESIAN_POINT('Ctrl Pts',(-20.1537425733231,17.6406134222842,
-19.584628618581));
#101683=CARTESIAN_POINT('Ctrl Pts',(-20.0721348493485,17.5675105048281,
-19.5778593740185));
#101684=CARTESIAN_POINT('Ctrl Pts',(-19.9931343333311,17.5062306342215,
-19.571351026869));
#101685=CARTESIAN_POINT('Ctrl Pts',(-19.7683195062158,17.3560189856748,
-19.5535366215855));
#101686=CARTESIAN_POINT('Ctrl Pts',(-19.6155670518583,17.2787399673944,
-19.5422128321443));
#101687=CARTESIAN_POINT('Ctrl Pts',(-19.427543704499,17.2106124556297,-19.5296790850231));
#101688=CARTESIAN_POINT('Ctrl Pts',(-19.3996982400038,17.2011743396427,
-19.5278545919433));
#101689=CARTESIAN_POINT('Ctrl Pts',(-19.3513391404719,17.1858985926629,
-19.524739673399));
#101690=CARTESIAN_POINT('Ctrl Pts',(-19.3309178131635,17.1797854616425,
-19.5234405163735));
#101691=CARTESIAN_POINT('Ctrl Pts',(-19.3017501179458,17.1715319942469,
-19.5216073163191));
#101692=CARTESIAN_POINT('Ctrl Pts',(-19.293077565758,17.16913756039,-19.5210650318227));
#101693=CARTESIAN_POINT('Ctrl Pts',(-19.278090262191,17.1651023121824,-19.520132620291));
#101694=CARTESIAN_POINT('Ctrl Pts',(-19.2717827567293,17.1634352829587,
-19.519741646839));
#101695=CARTESIAN_POINT('Ctrl Pts',(-19.259691302829,17.1602993236621,-19.5189948665447));
#101696=CARTESIAN_POINT('Ctrl Pts',(-19.2539086617314,17.1588256423046,
-19.5186389091404));
#101697=CARTESIAN_POINT('Ctrl Pts',(-19.2388562878887,17.1550573160074,
-19.5177153766906));
#101698=CARTESIAN_POINT('Ctrl Pts',(-19.2295770566492,17.1528008899165,
-19.5171490387924));
#101699=CARTESIAN_POINT('Ctrl Pts',(-19.1978869943889,17.1453215725636,
-19.5152248176217));
#101700=CARTESIAN_POINT('Ctrl Pts',(-19.1754059279767,17.1404012032832,
-19.5138766425967));
#101701=CARTESIAN_POINT('Ctrl Pts',(-18.981100328157,17.1011825799175,-19.5023583755693));
#101702=CARTESIAN_POINT('Ctrl Pts',(-18.8057153303756,17.0879710926004,
-19.4929364677679));
#101703=CARTESIAN_POINT('Ctrl Pts',(-18.543606155358,17.100776917375,-19.4786584615024));
#101704=CARTESIAN_POINT('Ctrl Pts',(-18.4568716572268,17.1104075240527,
-19.4738857159276));
#101705=CARTESIAN_POINT('Ctrl Pts',(-18.3336761093493,17.1318501841942,
-19.4667465262771));
#101706=CARTESIAN_POINT('Ctrl Pts',(-18.2965500849234,17.1393435745284,
-19.4645468137002));
#101707=CARTESIAN_POINT('Ctrl Pts',(-18.2522658486713,17.1495251446863,
-19.4618432947216));
#101708=CARTESIAN_POINT('Ctrl Pts',(-18.2448933202246,17.1512619041448,
-19.4613905333992));
#101709=CARTESIAN_POINT('Ctrl Pts',(-18.2334641924935,17.154019105174,-19.4606842684048));
#101710=CARTESIAN_POINT('Ctrl Pts',(-18.2294009441658,17.1550120894247,
-19.4604323175444));
#101711=CARTESIAN_POINT('Ctrl Pts',(-18.2218813668174,17.1568733715334,
-19.4599644071962));
#101712=CARTESIAN_POINT('Ctrl Pts',(-18.218424277394,17.1577383571726,-19.4597486397965));
#101713=CARTESIAN_POINT('Ctrl Pts',(-18.2106267385444,17.1597102852452,
-19.4592605129146));
#101714=CARTESIAN_POINT('Ctrl Pts',(-18.2062876338038,17.1608222705395,
-19.4589878666401));
#101715=CARTESIAN_POINT('Ctrl Pts',(-18.1935291856974,17.1641350732742,
-19.4581832634119));
#101716=CARTESIAN_POINT('Ctrl Pts',(-18.185119964687,17.1663740121364,-19.457649180118));
#101717=CARTESIAN_POINT('Ctrl Pts',(-18.1255636510094,17.1826246479992,
-19.45384111562));
#101718=CARTESIAN_POINT('Ctrl Pts',(-18.0749494120633,17.1985008914827,
-19.450471193311));
#101719=CARTESIAN_POINT('Ctrl Pts',(-18.0111255607433,17.2211864322055,
-19.4460944167734));
#101720=CARTESIAN_POINT('Ctrl Pts',(-17.9973136798349,17.2262585204482,
-19.4451394507847));
#101721=CARTESIAN_POINT('Ctrl Pts',(-17.8512337501419,17.2816378419006,
-19.4349634651908));
#101722=CARTESIAN_POINT('Ctrl Pts',(-17.7242725277974,17.34494304558,-19.4254871326029));
#101723=CARTESIAN_POINT('Ctrl Pts',(-17.5184301558905,17.4747823698172,
-19.4096959386094));
#101724=CARTESIAN_POINT('Ctrl Pts',(-17.4363125358383,17.5352690422902,
-19.4032524952369));
#101725=CARTESIAN_POINT('Ctrl Pts',(-17.3476244041252,17.6110406117418,
-19.3961392173745));
#101726=CARTESIAN_POINT('Ctrl Pts',(-17.3364906027865,17.6207563586093,
-19.3952430114356));
#101727=CARTESIAN_POINT('Ctrl Pts',(-17.3196645239569,17.6357525871239,
-19.393883415819));
#101728=CARTESIAN_POINT('Ctrl Pts',(-17.3138982253714,17.6409489808396,
-19.3934165329491));
#101729=CARTESIAN_POINT('Ctrl Pts',(-17.3034586776592,17.6504613147828,
-19.392569479121));
#101730=CARTESIAN_POINT('Ctrl Pts',(-17.2987760730753,17.6547668092685,
-19.3921888736617));
#101731=CARTESIAN_POINT('Ctrl Pts',(-17.2887080652307,17.6641080894601,
-19.3913690599734));
#101732=CARTESIAN_POINT('Ctrl Pts',(-17.2833294074414,17.6691510470874,
-19.390930164901));
#101733=CARTESIAN_POINT('Ctrl Pts',(-17.2688148935935,17.6829028475961,
-19.3897431864966));
#101734=CARTESIAN_POINT('Ctrl Pts',(-17.2597303057014,17.6916655463418,
-19.3889974350811));
#101735=CARTESIAN_POINT('Ctrl Pts',(-17.2159014219187,17.7347047404359,
-19.3853847861468));
#101736=CARTESIAN_POINT('Ctrl Pts',(-17.1822695630136,17.770096055695,-19.3825674146219));
#101737=CARTESIAN_POINT('Ctrl Pts',(-17.1228467552732,17.8371237459432,
-19.3774772542927));
#101738=CARTESIAN_POINT('Ctrl Pts',(-17.0966901564294,17.8684027185722,
-19.3751922462857));
#101739=CARTESIAN_POINT('Ctrl Pts',(-16.9982921795763,17.9932262243659,
-19.3663721453531));
#101740=CARTESIAN_POINT('Ctrl Pts',(-16.9330325132811,18.0919954830018,
-19.3600340072474));
#101741=CARTESIAN_POINT('Ctrl Pts',(-16.8405341843086,18.261234394413,-19.3494988692561));
#101742=CARTESIAN_POINT('Ctrl Pts',(-16.8082096184992,18.3286184553558,
-19.345375939591));
#101743=CARTESIAN_POINT('Ctrl Pts',(-16.7662504132167,18.4294359442087,
-19.3391195568939));
#101744=CARTESIAN_POINT('Ctrl Pts',(-16.7537679116808,18.4616260101356,
-19.3371091840047));
#101745=CARTESIAN_POINT('Ctrl Pts',(-16.7395821609449,18.5010416645928,
-19.3346157121536));
#101746=CARTESIAN_POINT('Ctrl Pts',(-16.7371218303058,18.5079915174602,
-19.3341748709852));
#101747=CARTESIAN_POINT('Ctrl Pts',(-16.7333370813812,18.518862718646,-19.3334832342328));
#101748=CARTESIAN_POINT('Ctrl Pts',(-16.731987748799,18.5227754178003,-19.3332338897752));
#101749=CARTESIAN_POINT('Ctrl Pts',(-16.7294965297472,18.5300686015429,
-19.3327683021498));
#101750=CARTESIAN_POINT('Ctrl Pts',(-16.7283517127724,18.5334480248905,
-19.332552235105));
#101751=CARTESIAN_POINT('Ctrl Pts',(-16.7257700044639,18.5411329334869,
-19.332060152502));
#101752=CARTESIAN_POINT('Ctrl Pts',(-16.7243384192817,18.5454401365259,
-19.3317838296685));
#101753=CARTESIAN_POINT('Ctrl Pts',(-16.7201156087495,18.5582831319594,
-19.3309584204669));
#101754=CARTESIAN_POINT('Ctrl Pts',(-16.7173648764901,18.5668319914621,
-19.3304070436378));
#101755=CARTESIAN_POINT('Ctrl Pts',(-16.6965145515918,18.633074244889,-19.3261209845785));
#101756=CARTESIAN_POINT('Ctrl Pts',(-16.6808415129951,18.6914964684959,
-19.3222617998779));
#101757=CARTESIAN_POINT('Ctrl Pts',(-16.6546073646064,18.8092124193351,
-19.314433419105));
#101758=CARTESIAN_POINT('Ctrl Pts',(-16.644031920348,18.8684508559508,-19.3104683957893));
#101759=CARTESIAN_POINT('Ctrl Pts',(-16.6214469210267,19.0359172690096,
-19.2993046531377));
#101760=CARTESIAN_POINT('Ctrl Pts',(-16.6152389138853,19.1447473494696,
-19.2921113262475));
#101761=CARTESIAN_POINT('Ctrl Pts',(-16.6189332628197,19.3283941239019,
-19.2803108674788));
#101762=CARTESIAN_POINT('Ctrl Pts',(-16.6244041523391,19.4030837634912,
-19.275603303176));
#101763=CARTESIAN_POINT('Ctrl Pts',(-16.6361829230597,19.4959652699098,
-19.2698679418007));
#101764=CARTESIAN_POINT('Ctrl Pts',(-16.638793470919,19.5145643746092,-19.268725302349));
#101765=CARTESIAN_POINT('Ctrl Pts',(-16.6429521100254,19.5415764842162,
-19.2670738846304));
#101766=CARTESIAN_POINT('Ctrl Pts',(-16.6443041714466,19.5500183439875,
-19.2665589317755));
#101767=CARTESIAN_POINT('Ctrl Pts',(-16.6467656960257,19.5648128637118,
-19.2656584203537));
#101768=CARTESIAN_POINT('Ctrl Pts',(-16.6478531088453,19.5711690327715,
-19.2652721675857));
#101769=CARTESIAN_POINT('Ctrl Pts',(-16.6500220358079,19.5835074492661,
-19.2645235809914));
#101770=CARTESIAN_POINT('Ctrl Pts',(-16.6511003077451,19.589490195629,-19.2641611482747));
#101771=CARTESIAN_POINT('Ctrl Pts',(-16.6537413168854,19.6037905732882,
-19.2632961065535));
#101772=CARTESIAN_POINT('Ctrl Pts',(-16.6553281975708,19.6121036824611,
-19.2627942698272));
#101773=CARTESIAN_POINT('Ctrl Pts',(-16.6612452408737,19.6421224712256,
-19.2609856718521));
#101774=CARTESIAN_POINT('Ctrl Pts',(-16.6658659759476,19.6637699081349,
-19.2596881687402));
#101775=CARTESIAN_POINT('Ctrl Pts',(-16.7123527334063,19.8659666151263,
-19.2476219094418));
#101776=CARTESIAN_POINT('Ctrl Pts',(-16.7774160942318,20.0403517913336,
-19.237707022582));
#101777=CARTESIAN_POINT('Ctrl Pts',(-16.9020317915031,20.2749691408593,
-19.2232256316142));
#101778=CARTESIAN_POINT('Ctrl Pts',(-16.9437034448167,20.3436844567665,
-19.2188098913474));
#101779=CARTESIAN_POINT('Ctrl Pts',(-17.0096018150903,20.4395931918922,
-19.2121539441067));
#101780=CARTESIAN_POINT('Ctrl Pts',(-17.0307858376637,20.4687962866522,
-19.2100557258158));
#101781=CARTESIAN_POINT('Ctrl Pts',(-17.0572426813734,20.5033736607171,
-19.2074647488007));
#101782=CARTESIAN_POINT('Ctrl Pts',(-17.0618126072333,20.5092812115193,
-19.2070182178698));
#101783=CARTESIAN_POINT('Ctrl Pts',(-17.068976302196,20.5184411614074,-19.2063195966805));
#101784=CARTESIAN_POINT('Ctrl Pts',(-17.071548611285,20.5217103739068,-19.2060690057086));
#101785=CARTESIAN_POINT('Ctrl Pts',(-17.0763437521366,20.5277678152197,
-19.2056023188159));
#101786=CARTESIAN_POINT('Ctrl Pts',(-17.0785639988411,20.5305580171941,
-19.2053864066902));
#101787=CARTESIAN_POINT('Ctrl Pts',(-17.0836082195718,20.5368643629984,
-19.2048962686192));
#101788=CARTESIAN_POINT('Ctrl Pts',(-17.0864363717232,20.540377082653,-19.2046217454134));
#101789=CARTESIAN_POINT('Ctrl Pts',(-17.0937669457726,20.5494227333948,
-19.2039109697467));
#101790=CARTESIAN_POINT('Ctrl Pts',(-17.0982861059209,20.5549419402853,
-19.2034735515306));
#101791=CARTESIAN_POINT('Ctrl Pts',(-17.1261965426133,20.5886793773029,
-19.20077725352));
#101792=CARTESIAN_POINT('Ctrl Pts',(-17.1502880085899,20.6163072188492,
-19.1984722199439));
#101793=CARTESIAN_POINT('Ctrl Pts',(-17.2905010253499,20.7689159230848,
-19.1852467127015));
#101794=CARTESIAN_POINT('Ctrl Pts',(-17.4206787319678,20.8801260208167,
-19.1737355294254));
#101795=CARTESIAN_POINT('Ctrl Pts',(-17.642208916033,21.0272514777714,-19.1564537798313));
#101796=CARTESIAN_POINT('Ctrl Pts',(-17.7251024988708,21.0745737921114,
-19.1503970165453));
#101797=CARTESIAN_POINT('Ctrl Pts',(-17.830159968478,21.1254763065328,-19.1432262657578));
#101798=CARTESIAN_POINT('Ctrl Pts',(-17.84954595053,21.1345091416212,-19.1419227555922));
#101799=CARTESIAN_POINT('Ctrl Pts',(-17.8772885830223,21.1469276084966,
-19.1400845366582));
#101800=CARTESIAN_POINT('Ctrl Pts',(-17.885534623554,21.1505557909514,-19.1395415249103));
#101801=CARTESIAN_POINT('Ctrl Pts',(-17.8997938349771,21.1567213739146,
-19.1386082557128));
#101802=CARTESIAN_POINT('Ctrl Pts',(-17.905795992482,21.1592837868447,-19.1382171477241));
#101803=CARTESIAN_POINT('Ctrl Pts',(-17.917306638786,21.1641350526862,-19.137470377294));
#101804=CARTESIAN_POINT('Ctrl Pts',(-17.9228131309953,21.166428455597,-19.1371145630072));
#101805=CARTESIAN_POINT('Ctrl Pts',(-17.937147490831,21.172327613964,-19.1361919781533));
#101806=CARTESIAN_POINT('Ctrl Pts',(-17.9459902214585,21.1758970772313,
-19.1356264396111));
#101807=CARTESIAN_POINT('Ctrl Pts',(-17.9761755332288,21.1878451557532,
-19.1337078903903));
#101808=CARTESIAN_POINT('Ctrl Pts',(-17.9976304466896,21.195936934427,-19.1323645092174));
#101809=CARTESIAN_POINT('Ctrl Pts',(-18.1851818948047,21.2632128522568,
-19.1207855173296));
#101810=CARTESIAN_POINT('Ctrl Pts',(-18.3579352619381,21.301779968253,-19.1113092300231));
#101811=CARTESIAN_POINT('Ctrl Pts',(-18.6195106265435,21.3266674229788,
-19.0970104506064));
#101812=CARTESIAN_POINT('Ctrl Pts',(-18.7059505313282,21.3295767221752,
-19.0922778542927));
#101813=CARTESIAN_POINT('Ctrl Pts',(-18.8299777535521,21.3261587560286,
-19.0851928046099));
#101814=CARTESIAN_POINT('Ctrl Pts',(-18.8675999548003,21.3241159337922,
-19.0830042089902));
#101815=CARTESIAN_POINT('Ctrl Pts',(-18.912683301989,21.3204592858548,-19.0803130120171));
#101816=CARTESIAN_POINT('Ctrl Pts',(-18.9202182271931,21.3198074755743,
-19.079860915993));
#101817=CARTESIAN_POINT('Ctrl Pts',(-18.9319122328687,21.3187327211717,
-19.0791554669945));
#101818=CARTESIAN_POINT('Ctrl Pts',(-18.9360739134314,21.3183378012635,
-19.0789036610764));
#101819=CARTESIAN_POINT('Ctrl Pts',(-18.943781348226,21.317583368309,-19.0784358822704));
#101820=CARTESIAN_POINT('Ctrl Pts',(-18.9473273745515,21.3172272271488,
-19.0782201005901));
#101821=CARTESIAN_POINT('Ctrl Pts',(-18.9553314382059,21.3164029276073,
-19.077731764547));
#101822=CARTESIAN_POINT('Ctrl Pts',(-18.9597888723646,21.3159295658945,
-19.0774589222978));
#101823=CARTESIAN_POINT('Ctrl Pts',(-18.9729100098262,21.3144939964824,
-19.0766532163828));
#101824=CARTESIAN_POINT('Ctrl Pts',(-18.981569189485,21.3134924438504,-19.076118217829));
#101825=CARTESIAN_POINT('Ctrl Pts',(-19.0431301354751,21.3059865082933,
-19.0722925744649));
#101826=CARTESIAN_POINT('Ctrl Pts',(-19.0957714001299,21.2975402777894,
-19.0689050266426));
#101827=CARTESIAN_POINT('Ctrl Pts',(-19.1656342010236,21.2836077891774,
-19.0643010877012));
#101828=CARTESIAN_POINT('Ctrl Pts',(-19.1831899234458,21.2798739735191,
-19.0631348875672));
#101829=CARTESIAN_POINT('Ctrl Pts',(-19.2477379940259,21.2652853487951,
-19.0588173024872));
#101830=CARTESIAN_POINT('Ctrl Pts',(-19.294402090412,21.2530490407273,-19.0556378676121));
#101831=CARTESIAN_POINT('Ctrl Pts',(-19.4453994711384,21.2078885063341,
-19.0452268413031));
#101832=CARTESIAN_POINT('Ctrl Pts',(-19.5476142114292,21.168469870797,-19.0379942682635));
#101833=CARTESIAN_POINT('Ctrl Pts',(-19.7146192688719,21.088711887975,-19.026098281523));
#101834=CARTESIAN_POINT('Ctrl Pts',(-19.7811164761318,21.0524574037317,
-19.0213354801221));
#101835=CARTESIAN_POINT('Ctrl Pts',(-19.8616162830218,21.0027944978295,
-19.0155405260873));
#101836=CARTESIAN_POINT('Ctrl Pts',(-19.8775637273199,20.9926587894657,
-19.0143908295255));
#101837=CARTESIAN_POINT('Ctrl Pts',(-19.9005445890706,20.9776171548102,
-19.0127311581586));
#101838=CARTESIAN_POINT('Ctrl Pts',(-19.9076869362773,20.9728800835885,
-19.0122149216488));
#101839=CARTESIAN_POINT('Ctrl Pts',(-19.9201552672233,20.9645011566095,
-19.0113129290612));
#101840=CARTESIAN_POINT('Ctrl Pts',(-19.9254936984965,20.9608781077735,
-19.0109264717404));
#101841=CARTESIAN_POINT('Ctrl Pts',(-19.9358248169164,20.9537974608059,
-19.0101780419633));
#101842=CARTESIAN_POINT('Ctrl Pts',(-19.9408193472458,20.9503426759105,
-19.0098159680157));
#101843=CARTESIAN_POINT('Ctrl Pts',(-19.9527191909723,20.9420354592015,
-19.0089526617102));
#101844=CARTESIAN_POINT('Ctrl Pts',(-19.9596105233162,20.9371631080892,
-19.0084521945275));
#101845=CARTESIAN_POINT('Ctrl Pts',(-19.9843471523556,20.9194508498627,
-19.0066536997101));
#101846=CARTESIAN_POINT('Ctrl Pts',(-20.0020217117558,20.9063740884316,
-19.0053647936434));
#101847=CARTESIAN_POINT('Ctrl Pts',(-20.167906501024,20.7795963401822,-18.9932204252046));
#101848=CARTESIAN_POINT('Ctrl Pts',(-20.3006547512269,20.6470296389423,
-18.9832348745875));
#101849=CARTESIAN_POINT('Ctrl Pts',(-20.4625580244662,20.4357743235519,
-18.9687215007074));
#101850=CARTESIAN_POINT('Ctrl Pts',(-20.5072417379585,20.3701362141873,
-18.9643555763264));
#101851=CARTESIAN_POINT('Ctrl Pts',(-20.5665927326588,20.2714600875568,
-18.9577673965023));
#101852=CARTESIAN_POINT('Ctrl Pts',(-20.5842696339808,20.2403073689867,
-18.9556838237881));
#101853=CARTESIAN_POINT('Ctrl Pts',(-20.6046593330345,20.202149943009,-18.9531090958991));
#101854=CARTESIAN_POINT('Ctrl Pts',(-20.6081371499621,20.1955580171731,
-18.9526634938179));
#101855=CARTESIAN_POINT('Ctrl Pts',(-20.6135001090306,20.1852615749484,
-18.951966012591));
#101856=CARTESIAN_POINT('Ctrl Pts',(-20.6154093115193,20.1815695637682,
-18.9517156248228));
#101857=CARTESIAN_POINT('Ctrl Pts',(-20.6189363572698,20.1746994587619,
-18.9512491186223));
#101858=CARTESIAN_POINT('Ctrl Pts',(-20.6205570474101,20.1715228909476,
-18.9510331827391));
#101859=CARTESIAN_POINT('Ctrl Pts',(-20.6242112024594,20.1643157872284,
-18.9505427344713));
#101860=CARTESIAN_POINT('Ctrl Pts',(-20.6262397957424,20.1602828527987,
-18.9502679232218));
#101861=CARTESIAN_POINT('Ctrl Pts',(-20.6322139864624,20.148310653789,-18.9494510988611));
#101862=CARTESIAN_POINT('Ctrl Pts',(-20.6361225704899,20.1403531732521,
-18.9489068637317));
#101863=CARTESIAN_POINT('Ctrl Pts',(-20.664856928934,20.0809122872286,-18.9448330223966));
#101864=CARTESIAN_POINT('Ctrl Pts',(-20.6876363959591,20.0284713799653,
-18.9411920729833));
#101865=CARTESIAN_POINT('Ctrl Pts',(-20.7683687191834,19.8198984997821,
-18.9267030292914));
#101866=CARTESIAN_POINT('Ctrl Pts',(-20.8099462681566,19.6580661827971,
-18.9155001930197));
#101867=CARTESIAN_POINT('Ctrl Pts',(-20.8399080762695,19.4351614982078,
-18.901006237287));
#101868=CARTESIAN_POINT('Ctrl Pts',(-20.8452891073375,19.3770014254749,
-18.8973012028165));
#101869=CARTESIAN_POINT('Ctrl Pts',(-20.8500786761297,19.2829677171489,
-18.8914415141523));
#101870=CARTESIAN_POINT('Ctrl Pts',(-20.8509926290775,19.2472045485215,
-18.8892430074392));
#101871=CARTESIAN_POINT('Ctrl Pts',(-20.8510022031418,19.2004601928484,
-18.8864069215302));
#101872=CARTESIAN_POINT('Ctrl Pts',(-20.8509191302474,19.1894867776335,
-18.8857438248984));
#101873=CARTESIAN_POINT('Ctrl Pts',(-20.8506443290511,19.1715808574569,
-18.8846660756149));
#101874=CARTESIAN_POINT('Ctrl Pts',(-20.8505038546913,19.1646478764242,
-18.8842498251253));
#101875=CARTESIAN_POINT('Ctrl Pts',(-20.8501671509485,19.1512747950672,
-18.8834488851803));
#101876=CARTESIAN_POINT('Ctrl Pts',(-20.8499755812812,19.1448346639406,
-18.8830640542783));
#101877=CARTESIAN_POINT('Ctrl Pts',(-20.84946265105,19.129887466604,-18.8821728824703));
#101878=CARTESIAN_POINT('Ctrl Pts',(-20.8491193700894,19.1213812264981,
-18.8816672336651));
#101879=CARTESIAN_POINT('Ctrl Pts',(-20.847863432152,19.0943134819767,-18.8800628357042));
#101880=CARTESIAN_POINT('Ctrl Pts',(-20.8467576609092,19.0757614989822,
-18.8789701371894));
#101881=CARTESIAN_POINT('Ctrl Pts',(-20.8436139219907,19.0325961004741,
-18.876442454687));
#101882=CARTESIAN_POINT('Ctrl Pts',(-20.8413892428455,19.0079987641029,
-18.8750132736541));
#101883=CARTESIAN_POINT('Ctrl Pts',(-20.8320826211675,18.9219185224895,
-18.8700446756409));
#101884=CARTESIAN_POINT('Ctrl Pts',(-20.8227356710758,18.8607101995958,
-18.8665718396773));
#101885=CARTESIAN_POINT('Ctrl Pts',(-20.7895029368918,18.6927921155633,
-18.8571028374997));
#101886=CARTESIAN_POINT('Ctrl Pts',(-20.7600278787111,18.5874456537938,
-18.8512348473893));
#101887=CARTESIAN_POINT('Ctrl Pts',(-20.7225806605155,18.4848898453927,
-18.8452754875981));
#101888=CARTESIAN_POINT('Origin',(-18.734,19.211,0.));
#101889=CARTESIAN_POINT('',(-20.7225806765445,18.484889889291,-18.0457834329553));
#101890=CARTESIAN_POINT('',(-20.7225806130935,18.4848897155193,-18.2676549617288));
#101891=CARTESIAN_POINT('',(-20.7225806137986,18.4848897174502,0.));
#101892=CARTESIAN_POINT('',(-20.8509999976816,19.2110990761722,-18.3109437209775));
#101893=CARTESIAN_POINT('Ctrl Pts',(-20.7225806130935,18.4848897155193,
-18.2676549617288));
#101894=CARTESIAN_POINT('Ctrl Pts',(-20.7253379764187,18.4924412395355,
-18.268103955216));
#101895=CARTESIAN_POINT('Ctrl Pts',(-20.7280524567443,18.5000088307141,
-18.2685519707272));
#101896=CARTESIAN_POINT('Ctrl Pts',(-20.7645972677333,18.6037465066057,
-18.2746683362838));
#101897=CARTESIAN_POINT('Ctrl Pts',(-20.7914816982396,18.70222490975,-18.2801721418135));
#101898=CARTESIAN_POINT('Ctrl Pts',(-20.8346080680977,18.9213865413653,
-18.2923170310514));
#101899=CARTESIAN_POINT('Ctrl Pts',(-20.8477551444556,19.0422954410914,
-18.2989530517298));
#101900=CARTESIAN_POINT('Ctrl Pts',(-20.85072784998,19.1751560966423,-18.3067847632183));
#101901=CARTESIAN_POINT('Ctrl Pts',(-20.8508914867126,19.1866690186424,
-18.3074678984705));
#101902=CARTESIAN_POINT('Ctrl Pts',(-20.8509827720571,19.2017457699954,
-18.3083690347001));
#101903=CARTESIAN_POINT('Ctrl Pts',(-20.8509953499484,19.205309144036,-18.308582495384));
#101904=CARTESIAN_POINT('Ctrl Pts',(-20.8509997172436,19.2096548902916,
-18.3088434247664));
#101905=CARTESIAN_POINT('Ctrl Pts',(-20.8510000697841,19.2104372756591,
-18.3088904248973));
#101906=CARTESIAN_POINT('Ctrl Pts',(-20.8509999886041,19.2112196594398,
-18.3089374488649));
#101907=CARTESIAN_POINT('Ctrl Pts',(-20.8509999976816,19.2110990761722,
-18.3109437209775));
#101908=CARTESIAN_POINT('Ctrl Pts',(-20.8509997507685,19.2163749670545,
-18.3112630160645));
#101909=CARTESIAN_POINT('Ctrl Pts',(-20.8509797813958,19.2216508039048,
-18.3115823111514));
#101910=CARTESIAN_POINT('Ctrl Pts',(-20.8509400905189,19.2269264921969,
-18.3119016062384));
#101911=CARTESIAN_POINT('Ctrl Pts',(-20.8503946018242,19.2994325325996,
-18.3162898151688));
#101912=CARTESIAN_POINT('Ctrl Pts',(-20.8461186979221,19.3720520465351,
-18.3206780240992));
#101913=CARTESIAN_POINT('Ctrl Pts',(-20.8380978239802,19.4443695505457,
-18.3250662330295));
#101914=CARTESIAN_POINT('Ctrl Pts',(-20.8300888543451,19.51657972339,-18.3294479291303));
#101915=CARTESIAN_POINT('Ctrl Pts',(-20.8183460011053,19.5884883006379,
-18.333829625231));
#101916=CARTESIAN_POINT('Ctrl Pts',(-20.8029067175876,19.6596802802896,
-18.3382113213318));
#101917=CARTESIAN_POINT('Ctrl Pts',(-20.7874855764568,19.7307886036995,
-18.3425878685909));
#101918=CARTESIAN_POINT('Ctrl Pts',(-20.7683767353654,19.8011815331898,
-18.3469644158501));
#101919=CARTESIAN_POINT('Ctrl Pts',(-20.7456691798644,19.870451371053,-18.3513409631092));
#101920=CARTESIAN_POINT('Ctrl Pts',(-20.722976025165,19.9396772789918,-18.3557147348257));
#101921=CARTESIAN_POINT('Ctrl Pts',(-20.696688834233,20.0077810512473,-18.3600885065421));
#101922=CARTESIAN_POINT('Ctrl Pts',(-20.6669468334595,20.0743687155665,
-18.3644622782586));
#101923=CARTESIAN_POINT('Ctrl Pts',(-20.6372138832767,20.140936117036,-18.3688347190216));
#101924=CARTESIAN_POINT('Ctrl Pts',(-20.6040284070354,20.2059878863297,
-18.3732071597847));
#101925=CARTESIAN_POINT('Ctrl Pts',(-20.5675776766823,20.2691502273176,
-18.3775796005477));
#101926=CARTESIAN_POINT('Ctrl Pts',(-20.5311260142799,20.3323141833736,
-18.3819521531146));
#101927=CARTESIAN_POINT('Ctrl Pts',(-20.4914091748394,20.3935881984054,
-18.3863247056814));
#101928=CARTESIAN_POINT('Ctrl Pts',(-20.4486594348613,20.4526247510585,
-18.3906972582483));
#101929=CARTESIAN_POINT('Ctrl Pts',(-20.4058653275905,20.5117225740729,
-18.3950743488151));
#101930=CARTESIAN_POINT('Ctrl Pts',(-20.3600323187904,20.5685779068974,
-18.3994514393819));
#101931=CARTESIAN_POINT('Ctrl Pts',(-20.3114344316434,20.6228745035823,
-18.4038285299488));
#101932=CARTESIAN_POINT('Ctrl Pts',(-20.2628100033865,20.677200753654,-18.4082080110072));
#101933=CARTESIAN_POINT('Ctrl Pts',(-20.2114180304767,20.7289651427762,
-18.4125874920657));
#101934=CARTESIAN_POINT('Ctrl Pts',(-20.1575691237185,20.7778886208009,
-18.4169669731242));
#101935=CARTESIAN_POINT('Ctrl Pts',(-20.1036247701345,20.8268988153621,
-18.4213542167834));
#101936=CARTESIAN_POINT('Ctrl Pts',(-20.0472151597967,20.8730577373941,
-18.4257414604427));
#101937=CARTESIAN_POINT('Ctrl Pts',(-19.9886831896891,20.9161272953981,
-18.4301287041019));
#101938=CARTESIAN_POINT('Ctrl Pts',(-19.9488870900788,20.9454104447154,
-18.4331116070412));
#101939=CARTESIAN_POINT('Ctrl Pts',(-19.9081105258029,20.973266366868,-18.4360945099806));
#101940=CARTESIAN_POINT('Ctrl Pts',(-19.8664678605233,20.9996323112596,
-18.4390774129199));
#101941=CARTESIAN_POINT('Ctrl Pts',(-19.8052064921927,21.0384197860745,
-18.4434656218502));
#101942=CARTESIAN_POINT('Ctrl Pts',(-19.7418305075797,21.0741319931224,
-18.4478538307805));
#101943=CARTESIAN_POINT('Ctrl Pts',(-19.6766813842659,21.1065318007774,
-18.4522420397107));
#101944=CARTESIAN_POINT('Ctrl Pts',(-19.6116289530531,21.1388835217459,
-18.4566237358114));
#101945=CARTESIAN_POINT('Ctrl Pts',(-19.5448090356318,21.1679323895269,
-18.461005431912));
#101946=CARTESIAN_POINT('Ctrl Pts',(-19.4765908557838,21.1934852637299,
-18.4653871280127));
#101947=CARTESIAN_POINT('Ctrl Pts',(-19.4084528377262,21.2190081112721,
-18.4697636752717));
#101948=CARTESIAN_POINT('Ctrl Pts',(-19.3389202706957,21.2410429575789,
-18.4741402225307));
#101949=CARTESIAN_POINT('Ctrl Pts',(-19.2683841301352,21.2594439463797,
-18.4785167697897));
#101950=CARTESIAN_POINT('Ctrl Pts',(-19.1978927225701,21.2778332655408,
-18.482890541506));
#101951=CARTESIAN_POINT('Ctrl Pts',(-19.1263994698862,21.2925931782368,
-18.4872643132223));
#101952=CARTESIAN_POINT('Ctrl Pts',(-19.0543110010058,21.3036275021214,
-18.4916380849387));
#101953=CARTESIAN_POINT('Ctrl Pts',(-18.9822444688885,21.3146584682241,
-18.4960105257016));
#101954=CARTESIAN_POINT('Ctrl Pts',(-18.9095835567039,21.3219660233356,
-18.5003829664645));
#101955=CARTESIAN_POINT('Ctrl Pts',(-18.8367439345953,21.3255053047708,
-18.5047554072274));
#101956=CARTESIAN_POINT('Ctrl Pts',(-18.7639024499697,21.3290446767058,
-18.5091279597941));
#101957=CARTESIAN_POINT('Ctrl Pts',(-18.6908827282539,21.3288155622467,
-18.5135005123608));
#101958=CARTESIAN_POINT('Ctrl Pts',(-18.6181027067747,21.3248251624538,
-18.5178730649275));
#101959=CARTESIAN_POINT('Ctrl Pts',(-18.545247151444,21.3208306212736,-18.5222501554941));
#101960=CARTESIAN_POINT('Ctrl Pts',(-18.4726322757206,21.3130670274164,
-18.5266272460608));
#101961=CARTESIAN_POINT('Ctrl Pts',(-18.4006723159525,21.3015936130792,
-18.5310043366275));
#101962=CARTESIAN_POINT('Ctrl Pts',(-18.3286730561795,21.2901139326845,
-18.5353838176858));
#101963=CARTESIAN_POINT('Ctrl Pts',(-18.2573298966116,21.274920498468,-18.5397632987441));
#101964=CARTESIAN_POINT('Ctrl Pts',(-18.1870456019999,21.2561234404085,
-18.5441427798024));
#101965=CARTESIAN_POINT('Ctrl Pts',(-18.1166367289477,21.2372930646898,
-18.5485300234614));
#101966=CARTESIAN_POINT('Ctrl Pts',(-18.0472909281451,21.2148464584352,
-18.5529172671205));
#101967=CARTESIAN_POINT('Ctrl Pts',(-17.9793940004978,21.1889430693312,
-18.5573045107796));
#101968=CARTESIAN_POINT('Ctrl Pts',(-17.9332306321345,21.1713312607487,
-18.5602874137201));
#101969=CARTESIAN_POINT('Ctrl Pts',(-17.8877366290261,21.1521225055481,
-18.5632703166607));
#101970=CARTESIAN_POINT('Ctrl Pts',(-17.8430266573749,21.1313789997632,
-18.5662532196012));
#101971=CARTESIAN_POINT('Ctrl Pts',(-17.7772529124848,21.1008628082464,
-18.5706414285354));
#101972=CARTESIAN_POINT('Ctrl Pts',(-17.7129203794324,21.0669039749608,
-18.5750296374695));
#101973=CARTESIAN_POINT('Ctrl Pts',(-17.6504132837269,21.0296612736616,
-18.5794178464036));
#101974=CARTESIAN_POINT('Ctrl Pts',(-17.587998958915,20.992473846706,-18.5837995425081));
#101975=CARTESIAN_POINT('Ctrl Pts',(-17.5274051041887,20.9520124717683,
-18.5881812386125));
#101976=CARTESIAN_POINT('Ctrl Pts',(-17.4689939738821,20.9084830643884,
-18.592562934717));
#101977=CARTESIAN_POINT('Ctrl Pts',(-17.4106514813021,20.8650048075263,
-18.5969394819799));
#101978=CARTESIAN_POINT('Ctrl Pts',(-17.3544870028684,20.8184659667525,
-18.6013160292428));
#101979=CARTESIAN_POINT('Ctrl Pts',(-17.3008348082146,20.7691163413092,
-18.6056925765056));
#101980=CARTESIAN_POINT('Ctrl Pts',(-17.2472166390029,20.7197980126811,
-18.6100663482258));
#101981=CARTESIAN_POINT('Ctrl Pts',(-17.1961079465062,20.6676727619676,
-18.614440119946));
#101982=CARTESIAN_POINT('Ctrl Pts',(-17.1478097053802,20.6130304380626,
-18.6188138916662));
#101983=CARTESIAN_POINT('Ctrl Pts',(-17.0995261615713,20.5584047420004,
-18.6231863324329));
#101984=CARTESIAN_POINT('Ctrl Pts',(-17.0540516905116,20.5012638546118,
-18.6275587731997));
#101985=CARTESIAN_POINT('Ctrl Pts',(-17.0116490089849,20.4419330053863,
-18.6319312139665));
#101986=CARTESIAN_POINT('Ctrl Pts',(-16.9692452432171,20.3826006390646,
-18.636303766537));
#101987=CARTESIAN_POINT('Ctrl Pts',(-16.9299137017802,20.3210785933442,
-18.6406763191075));
#101988=CARTESIAN_POINT('Ctrl Pts',(-16.8938745512703,20.257722185175,-18.6450488716781));
#101989=CARTESIAN_POINT('Ctrl Pts',(-16.8577979979711,20.1943000233362,
-18.6494259622486));
#101990=CARTESIAN_POINT('Ctrl Pts',(-16.8250208968201,20.1290401182288,
-18.653803052819));
#101991=CARTESIAN_POINT('Ctrl Pts',(-16.7957176611923,20.0623228383323,
-18.6581801433895));
#101992=CARTESIAN_POINT('Ctrl Pts',(-16.76639842198,19.9955691216533,-18.6625596244516));
#101993=CARTESIAN_POINT('Ctrl Pts',(-16.7405569966209,19.9273568969086,
-18.6669391055137));
#101994=CARTESIAN_POINT('Ctrl Pts',(-16.718318792152,19.8580844367843,-18.6713185865757));
#101995=CARTESIAN_POINT('Ctrl Pts',(-16.6960411706153,19.7886891916906,
-18.6757058302385));
#101996=CARTESIAN_POINT('Ctrl Pts',(-16.6773796475306,19.7182304251215,
-18.6800930739013));
#101997=CARTESIAN_POINT('Ctrl Pts',(-16.66240897934,19.6471188405936,-18.6844803175641));
#101998=CARTESIAN_POINT('Ctrl Pts',(-16.6522303676452,19.5987698159082,
-18.6874632204703));
#101999=CARTESIAN_POINT('Ctrl Pts',(-16.6437568500118,19.5501192245646,
-18.6904461233765));
#102000=CARTESIAN_POINT('Ctrl Pts',(-16.6369981960583,19.5012971482211,
-18.6934290262827));
#102001=CARTESIAN_POINT('Ctrl Pts',(-16.6270554032346,19.4294740021261,
-18.6978172352092));
#102002=CARTESIAN_POINT('Ctrl Pts',(-16.6207874279489,19.3569992504147,
-18.7022054441356));
#102003=CARTESIAN_POINT('Ctrl Pts',(-16.6182687405808,19.2842819071561,
-18.7065936530621));
#102004=CARTESIAN_POINT('Ctrl Pts',(-16.6157537913624,19.2116724884915,
-18.7109753491589));
#102005=CARTESIAN_POINT('Ctrl Pts',(-16.6169771002007,19.1388216711239,
-18.7153570452558));
#102006=CARTESIAN_POINT('Ctrl Pts',(-16.6219616061144,19.0661455117954,
-18.7197387413526));
#102007=CARTESIAN_POINT('Ctrl Pts',(-16.6269402548369,18.9935547527373,
-18.7241152886079));
#102008=CARTESIAN_POINT('Ctrl Pts',(-16.635671288018,18.9211387228721,-18.7284918358631));
#102009=CARTESIAN_POINT('Ctrl Pts',(-16.6481255978396,18.8493137016531,
-18.7328683831184));
#102010=CARTESIAN_POINT('Ctrl Pts',(-16.6605720093189,18.7775342308183,
-18.737242154831));
#102011=CARTESIAN_POINT('Ctrl Pts',(-16.6767369302059,18.706345499076,-18.7416159265436));
#102012=CARTESIAN_POINT('Ctrl Pts',(-16.6965395553235,18.6361574681891,
-18.7459896982562));
#102013=CARTESIAN_POINT('Ctrl Pts',(-16.7163361544359,18.5659907957552,
-18.7503621390155));
#102014=CARTESIAN_POINT('Ctrl Pts',(-16.7397681292067,18.4968246835922,
-18.7547345797747));
#102015=CARTESIAN_POINT('Ctrl Pts',(-16.7667042167163,18.4290560754925,
-18.7591070205339));
#102016=CARTESIAN_POINT('Ctrl Pts',(-16.793640992985,18.3612857345413,-18.763479573097));
#102017=CARTESIAN_POINT('Ctrl Pts',(-16.8240818798548,18.2949134161282,
-18.7678521256601));
#102018=CARTESIAN_POINT('Ctrl Pts',(-16.8578472840042,18.2303165718431,
-18.7722246782231));
#102019=CARTESIAN_POINT('Ctrl Pts',(-16.8916477311643,18.1656526865152,
-18.7766017687863));
#102020=CARTESIAN_POINT('Ctrl Pts',(-16.9287793604438,18.1027683827113,
-18.7809788593494));
#102021=CARTESIAN_POINT('Ctrl Pts',(-16.9690167487982,18.0420162007209,
-18.7853559499125));
#102022=CARTESIAN_POINT('Ctrl Pts',(-17.0092761122842,17.9812308397084,
-18.7897354309673));
#102023=CARTESIAN_POINT('Ctrl Pts',(-17.0526443249076,17.922580307009,-18.7941149120221));
#102024=CARTESIAN_POINT('Ctrl Pts',(-17.0988543828187,17.866385627545,-18.7984943930769));
#102025=CARTESIAN_POINT('Ctrl Pts',(-17.1451463477484,17.8100913433872,
-18.8028816367326));
#102026=CARTESIAN_POINT('Ctrl Pts',(-17.1942898914324,17.756261961755,-18.8072688803883));
#102027=CARTESIAN_POINT('Ctrl Pts',(-17.2459801414532,17.7051826470085,
-18.811656124044));
#102028=CARTESIAN_POINT('Ctrl Pts',(-17.2811245310937,17.6704536344907,
-18.8146390270174));
#102029=CARTESIAN_POINT('Ctrl Pts',(-17.3174454256991,17.6369951039856,
-18.8176219299908));
#102030=CARTESIAN_POINT('Ctrl Pts',(-17.3548387352822,17.6048856809362,
-18.8206048329642));
#102031=CARTESIAN_POINT('Ctrl Pts',(-17.4098487897262,17.5576488589001,
-18.8249930418924));
#102032=CARTESIAN_POINT('Ctrl Pts',(-17.4673958504111,17.5131492751001,
-18.8293812508206));
#102033=CARTESIAN_POINT('Ctrl Pts',(-17.5271763106366,17.4716709388988,
-18.8337694597489));
#102034=CARTESIAN_POINT('Ctrl Pts',(-17.5868680467466,17.4302541634261,
-18.8381511558474));
#102035=CARTESIAN_POINT('Ctrl Pts',(-17.6487862091493,17.3918500068484,
-18.8425328519459));
#102036=CARTESIAN_POINT('Ctrl Pts',(-17.7125933764228,17.3567029608737,
-18.8469145480444));
#102037=CARTESIAN_POINT('Ctrl Pts',(-17.7763255651959,17.3215972154757,
-18.8512910953013));
#102038=CARTESIAN_POINT('Ctrl Pts',(-17.8419419289082,17.2897412091786,
-18.8556676425581));
#102039=CARTESIAN_POINT('Ctrl Pts',(-17.9090766869075,17.261335791087,-18.8600441898149));
#102040=CARTESIAN_POINT('Ctrl Pts',(-17.9761688690183,17.232948387299,-18.8644179615291));
#102041=CARTESIAN_POINT('Ctrl Pts',(-18.0447770916552,17.2080074173236,
-18.8687917332432));
#102042=CARTESIAN_POINT('Ctrl Pts',(-18.1145129035437,17.1866668413218,
-18.8731655049573));
#102043=CARTESIAN_POINT('Ctrl Pts',(-18.1842274945899,17.165332759329,-18.877537945718));
#102044=CARTESIAN_POINT('Ctrl Pts',(-18.255068532685,17.1475970372532,-18.8819103864787));
#102045=CARTESIAN_POINT('Ctrl Pts',(-18.3266312007886,17.1335641618984,
-18.8862828272393));
#102046=CARTESIAN_POINT('Ctrl Pts',(-18.3981956987569,17.1195309277215,
-18.8906553798038));
#102047=CARTESIAN_POINT('Ctrl Pts',(-18.4704813896214,17.1092008191085,
-18.8950279323682));
#102048=CARTESIAN_POINT('Ctrl Pts',(-18.5430736858689,17.1026271338844,
-18.8994004849326));
#102049=CARTESIAN_POINT('Ctrl Pts',(-18.6157413211391,17.0960466262419,
-18.903777575497));
#102050=CARTESIAN_POINT('Ctrl Pts',(-18.6887157156737,17.0932303693191,
-18.9081546660613));
#102051=CARTESIAN_POINT('Ctrl Pts',(-18.7615784216612,17.0941796413822,
-18.9125317566257));
#102052=CARTESIAN_POINT('Ctrl Pts',(-18.8344809206765,17.0951294318781,
-18.9169112376817));
#102053=CARTESIAN_POINT('Ctrl Pts',(-18.9072711279992,17.0998488145901,
-18.9212907187377));
#102054=CARTESIAN_POINT('Ctrl Pts',(-18.9795345883529,17.1082870462371,
-18.9256701997936));
#102055=CARTESIAN_POINT('Ctrl Pts',(-19.0519261352051,17.116740234593,-18.9300574434504));
#102056=CARTESIAN_POINT('Ctrl Pts',(-19.1237885946081,17.1289253543979,
-18.9344446871071));
#102057=CARTESIAN_POINT('Ctrl Pts',(-19.194717166806,17.1447404102557,-18.9388319307639));
#102058=CARTESIAN_POINT('Ctrl Pts',(-19.2429417616886,17.155493124404,-18.9418148337244));
#102059=CARTESIAN_POINT('Ctrl Pts',(-19.2907349020838,17.1679227808446,
-18.944797736685));
#102060=CARTESIAN_POINT('Ctrl Pts',(-19.3379741345028,17.1819844148328,
-18.9477806396456));
#102061=CARTESIAN_POINT('Ctrl Pts',(-19.407471955745,17.2026717307615,-18.9521690525414));
#102062=CARTESIAN_POINT('Ctrl Pts',(-19.4760413397733,17.2269742190327,
-18.9565574654372));
#102063=CARTESIAN_POINT('Ctrl Pts',(-19.5432790871371,17.2547903079878,
-18.960945878333));
#102064=CARTESIAN_POINT('Ctrl Pts',(-19.6105530590736,17.2826213829585,
-18.9653366555017));
#102065=CARTESIAN_POINT('Ctrl Pts',(-19.6764934827205,17.3139697486589,
-18.9697274326704));
#102066=CARTESIAN_POINT('Ctrl Pts',(-19.7407097395332,17.3486830290391,
-18.9741182098391));
#102067=CARTESIAN_POINT('Ctrl Pts',(-19.8047168505583,17.3832832518117,
-18.9784946866952));
#102068=CARTESIAN_POINT('Ctrl Pts',(-19.8670105658331,17.4212263095738,
-18.9828711635512));
#102069=CARTESIAN_POINT('Ctrl Pts',(-19.9272240799091,17.4623132655833,
-18.9872476404073));
#102070=CARTESIAN_POINT('Ctrl Pts',(-19.9873983214049,17.5033734237751,
-18.9916212628287));
#102071=CARTESIAN_POINT('Ctrl Pts',(-20.0454946569097,17.5475731395301,
-18.9959948852502));
#102072=CARTESIAN_POINT('Ctrl Pts',(-20.1011734655357,17.5946690576694,
-19.0003685076716));
#102073=CARTESIAN_POINT('Ctrl Pts',(-20.1568343267224,17.641749794968,-19.0047407203049));
#102074=CARTESIAN_POINT('Ctrl Pts',(-20.2100788408593,17.69172456909,-19.0091129329383));
#102075=CARTESIAN_POINT('Ctrl Pts',(-20.260600151433,17.7443095153903,-19.0134851455716));
#102076=CARTESIAN_POINT('Ctrl Pts',(-20.3114804721155,17.7972681362267,
-19.0178884276391));
#102077=CARTESIAN_POINT('Ctrl Pts',(-20.3595983637694,17.8528738414539,
-19.0222917097066));
#102078=CARTESIAN_POINT('Ctrl Pts',(-20.4046791157894,17.9107999030667,
-19.0266949917741));
#102079=CARTESIAN_POINT('Ctrl Pts',(-20.4494793907307,17.9683655684614,
-19.031070878121));
#102080=CARTESIAN_POINT('Ctrl Pts',(-20.4912799667756,18.0282223741802,
-19.0354467644678));
#102081=CARTESIAN_POINT('Ctrl Pts',(-20.529853854989,18.0900192100124,-19.0398226508146));
#102082=CARTESIAN_POINT('Ctrl Pts',(-20.5687899873458,18.152396374738,-19.0442396307425));
#102083=CARTESIAN_POINT('Ctrl Pts',(-20.6044382512207,18.2167497689265,
-19.0486566106703));
#102084=CARTESIAN_POINT('Ctrl Pts',(-20.636612911253,18.2826934181353,-19.0530735905982));
#102085=CARTESIAN_POINT('Ctrl Pts',(-20.6687875712854,18.3486370673441,
-19.057490570526));
#102086=CARTESIAN_POINT('Ctrl Pts',(-20.6974884771346,18.4161704915587,
-19.0619075504539));
#102087=CARTESIAN_POINT('Ctrl Pts',(-20.7225806137985,18.4848897174502,
-19.0663245303817));
#102088=CARTESIAN_POINT('',(-20.8509990913971,19.2090541452052,-18.0890148351743));
#102089=CARTESIAN_POINT('Ctrl Pts',(-20.7225806605155,18.4848898453927,
-18.8452754875981));
#102090=CARTESIAN_POINT('Ctrl Pts',(-20.7113123812129,18.4540296760972,
-18.843482250775));
#102091=CARTESIAN_POINT('Ctrl Pts',(-20.6993222446765,18.4234222395519,
-18.8416799355164));
#102092=CARTESIAN_POINT('Ctrl Pts',(-20.6575319528,18.3236548005616,-18.8356910254822));
#102093=CARTESIAN_POINT('Ctrl Pts',(-20.6247656769741,18.2558249992468,
-18.8314363670982));
#102094=CARTESIAN_POINT('Ctrl Pts',(-20.5838856248111,18.1815816305726,
-18.8264132177367));
#102095=CARTESIAN_POINT('Ctrl Pts',(-20.5792539498844,18.1733021359491,
-18.8258477181026));
#102096=CARTESIAN_POINT('Ctrl Pts',(-20.5723045746278,18.1610732133138,
-18.8250041205476));
#102097=CARTESIAN_POINT('Ctrl Pts',(-20.5700293834158,18.1570995925474,
-18.8247286884852));
#102098=CARTESIAN_POINT('Ctrl Pts',(-20.5659565723776,18.1500396455026,
-18.8242369226343));
#102099=CARTESIAN_POINT('Ctrl Pts',(-20.5641640160301,18.1469504564686,
-18.8240209171774));
#102100=CARTESIAN_POINT('Ctrl Pts',(-20.5602911440827,18.1403149105042,
-18.8235551451304));
#102101=CARTESIAN_POINT('Ctrl Pts',(-20.5582083430706,18.1367701250521,
-18.8233052224583));
#102102=CARTESIAN_POINT('Ctrl Pts',(-20.5524255485203,18.1269935192338,
-18.8226129291748));
#102103=CARTESIAN_POINT('Ctrl Pts',(-20.5487038996259,18.1207746659344,
-18.8221691841879));
#102104=CARTESIAN_POINT('Ctrl Pts',(-20.5280542387278,18.0866678935757,
-18.8197173785031));
#102105=CARTESIAN_POINT('Ctrl Pts',(-20.5105162385413,18.0591566599313,
-18.8176727794783));
#102106=CARTESIAN_POINT('Ctrl Pts',(-20.4017836244343,17.8969850172192,
-18.8052648880665));
#102107=CARTESIAN_POINT('Ctrl Pts',(-20.295956086838,17.7727960098617,-18.7943130933028));
#102108=CARTESIAN_POINT('Ctrl Pts',(-20.0915016564241,17.5823449808717,
-18.7760620014946));
#102109=CARTESIAN_POINT('Ctrl Pts',(-19.9995963204598,17.5099410141166,
-18.7686228828945));
#102110=CARTESIAN_POINT('Ctrl Pts',(-19.8902556624036,17.4375947956546,
-18.7606174281779));
#102111=CARTESIAN_POINT('Ctrl Pts',(-19.8782592760728,17.4298307490648,
-18.7597494731479));
#102112=CARTESIAN_POINT('Ctrl Pts',(-19.859041198722,17.4176671312054,-18.7583751914239));
#102113=CARTESIAN_POINT('Ctrl Pts',(-19.8518703321578,17.4131884412315,
-18.7578659368403));
#102114=CARTESIAN_POINT('Ctrl Pts',(-19.8391760175082,17.4053653029108,
-18.756970565691));
#102115=CARTESIAN_POINT('Ctrl Pts',(-19.833663773927,17.4020029644157,-18.7565837930307));
#102116=CARTESIAN_POINT('Ctrl Pts',(-19.8222308203897,17.3951007006677,
-18.755785722893));
#102117=CARTESIAN_POINT('Ctrl Pts',(-19.8163080118224,17.3915643861245,
-18.7553745608133));
#102118=CARTESIAN_POINT('Ctrl Pts',(-19.8010605116558,17.382561405085,-18.7543218379008));
#102119=CARTESIAN_POINT('Ctrl Pts',(-19.7917109736051,17.3771370460735,
-18.753681818445));
#102120=CARTESIAN_POINT('Ctrl Pts',(-19.7525150425459,17.3547960620988,
-18.7510210498005));
#102121=CARTESIAN_POINT('Ctrl Pts',(-19.7223002266858,17.3385340298066,
-18.7490238316801));
#102122=CARTESIAN_POINT('Ctrl Pts',(-19.6425552085979,17.2980824952101,
-18.7438794698669));
#102123=CARTESIAN_POINT('Ctrl Pts',(-19.5924512962847,17.2750795562293,
-18.7407717208731));
#102124=CARTESIAN_POINT('Ctrl Pts',(-19.4404219898909,17.2123468928775,
-18.7316269788336));
#102125=CARTESIAN_POINT('Ctrl Pts',(-19.3362575503628,17.1785303208363,
-18.7257387140683));
#102126=CARTESIAN_POINT('Ctrl Pts',(-19.185213426797,17.142132491777,-18.7172798297436));
#102127=CARTESIAN_POINT('Ctrl Pts',(-19.1401412152453,17.1328143986246,
-18.7147637885898));
#102128=CARTESIAN_POINT('Ctrl Pts',(-19.0730014604782,17.1212017992091,
-18.7109849046902));
#102129=CARTESIAN_POINT('Ctrl Pts',(-19.0511430224418,17.117773121191,-18.7097497768155));
#102130=CARTESIAN_POINT('Ctrl Pts',(-18.9782541198754,17.1075077681755,
-18.7056036522646));
#102131=CARTESIAN_POINT('Ctrl Pts',(-18.9270322243903,17.1021905540812,
-18.7026454778712));
#102132=CARTESIAN_POINT('Ctrl Pts',(-18.867052076745,17.0981675916767,-18.6990775024238));
#102133=CARTESIAN_POINT('Ctrl Pts',(-18.8584286626431,17.0976422113308,
-18.6985620256782));
#102134=CARTESIAN_POINT('Ctrl Pts',(-18.8453433190052,17.0969253540233,
-18.6977757076402));
#102135=CARTESIAN_POINT('Ctrl Pts',(-18.8408834816923,17.0966951818743,
-18.6975069832111));
#102136=CARTESIAN_POINT('Ctrl Pts',(-18.8328642849029,17.0963067486482,
-18.6970224336897));
#102137=CARTESIAN_POINT('Ctrl Pts',(-18.8293052282903,17.0961433601086,
-18.6968068987933));
#102138=CARTESIAN_POINT('Ctrl Pts',(-18.821556239394,17.0958072215883,-18.696336559941));
#102139=CARTESIAN_POINT('Ctrl Pts',(-18.8173662547135,17.0956379383725,
-18.6960815698099));
#102140=CARTESIAN_POINT('Ctrl Pts',(-18.8055579713674,17.0951959991779,
-18.6953611135334));
#102141=CARTESIAN_POINT('Ctrl Pts',(-18.7979387537046,17.0949520457045,
-18.6948940874485));
#102142=CARTESIAN_POINT('Ctrl Pts',(-18.7515938608364,17.093718696713,-18.6920409088379));
#102143=CARTESIAN_POINT('Ctrl Pts',(-18.712850946846,17.0937513276122,-18.6896030499337));
#102144=CARTESIAN_POINT('Ctrl Pts',(-18.5834929022021,17.0974108849747,
-18.6813344256672));
#102145=CARTESIAN_POINT('Ctrl Pts',(-18.4931159169131,17.105795927002,-18.6753498012045));
#102146=CARTESIAN_POINT('Ctrl Pts',(-18.3372635874928,17.1304245151083,
-18.6649228875809));
#102147=CARTESIAN_POINT('Ctrl Pts',(-18.2714997253667,17.1440485806457,
-18.6604883537513));
#102148=CARTESIAN_POINT('Ctrl Pts',(-18.0953557075175,17.1893690885935,
-18.6486171010104));
#102149=CARTESIAN_POINT('Ctrl Pts',(-17.9867142930103,17.2269562587735,
-18.641313125844));
#102150=CARTESIAN_POINT('Ctrl Pts',(-17.868588098506,17.2789144507888,-18.6334337531152));
#102151=CARTESIAN_POINT('Ctrl Pts',(-17.8555937025524,17.2847874673492,
-18.6325676243562));
#102152=CARTESIAN_POINT('Ctrl Pts',(-17.8349986740339,17.2943474629822,
-18.6311956787686));
#102153=CARTESIAN_POINT('Ctrl Pts',(-17.8273592287719,17.297949334983,-18.6306869495171));
#102154=CARTESIAN_POINT('Ctrl Pts',(-17.8139191786754,17.3043846866594,
-18.6297921892407));
#102155=CARTESIAN_POINT('Ctrl Pts',(-17.8081096339815,17.3071991431927,
-18.6294055049388));
#102156=CARTESIAN_POINT('Ctrl Pts',(-17.7961157072515,17.3130775343609,
-18.6286073172593));
#102157=CARTESIAN_POINT('Ctrl Pts',(-17.7899332461023,17.3161452303458,
-18.6281959507582));
#102158=CARTESIAN_POINT('Ctrl Pts',(-17.7740927630202,17.3241019442315,
-18.6271420829112));
#102159=CARTESIAN_POINT('Ctrl Pts',(-17.7644569619894,17.3290349417425,
-18.6265011295292));
#102160=CARTESIAN_POINT('Ctrl Pts',(-17.724319012616,17.34997344661,-18.6238312679306));
#102161=CARTESIAN_POINT('Ctrl Pts',(-17.6941709566264,17.366648816462,-18.6218260965537));
#102162=CARTESIAN_POINT('Ctrl Pts',(-17.6166178156028,17.4120511171355,
-18.6166565980664));
#102163=CARTESIAN_POINT('Ctrl Pts',(-17.5699093038678,17.441917318193,-18.6135321724689));
#102164=CARTESIAN_POINT('Ctrl Pts',(-17.4344715393567,17.536208068346,-18.6043583487418));
#102165=CARTESIAN_POINT('Ctrl Pts',(-17.3495159790017,17.6057252311954,
-18.5984575786685));
#102166=CARTESIAN_POINT('Ctrl Pts',(-17.2253112073214,17.7245851535917,
-18.5890964014264));
#102167=CARTESIAN_POINT('Ctrl Pts',(-17.1822224217581,17.76962684187,-18.5856839902293));
#102168=CARTESIAN_POINT('Ctrl Pts',(-17.1041153451539,17.8588417505782,
-18.5790314238806));
#102169=CARTESIAN_POINT('Ctrl Pts',(-17.0687523206251,17.9026403749648,
-18.5758089764813));
#102170=CARTESIAN_POINT('Ctrl Pts',(-17.029908573929,17.9548792126231,-18.5719467462809));
#102171=CARTESIAN_POINT('Ctrl Pts',(-17.0246824943781,17.9620001282147,
-18.5714198751705));
#102172=CARTESIAN_POINT('Ctrl Pts',(-17.0168571441804,17.9728038404035,
-18.5706195801113));
#102173=CARTESIAN_POINT('Ctrl Pts',(-17.0142247480488,17.9764626782294,
-18.5703483875093));
#102174=CARTESIAN_POINT('Ctrl Pts',(-17.0095309312963,17.9830308859647,
-18.5698612109275));
#102175=CARTESIAN_POINT('Ctrl Pts',(-17.0074651589293,17.9859370807053,
-18.5696455312086));
#102176=CARTESIAN_POINT('Ctrl Pts',(-17.0030041910248,17.992246608846,-18.5691770011826));
#102177=CARTESIAN_POINT('Ctrl Pts',(-17.0006117183176,17.9956517439941,
-18.5689239762789));
#102178=CARTESIAN_POINT('Ctrl Pts',(-16.9939490143187,18.0051942652536,
-18.5682144840628));
#102179=CARTESIAN_POINT('Ctrl Pts',(-16.9897012831795,18.0113471813133,
-18.5677565303065));
#102180=CARTESIAN_POINT('Ctrl Pts',(-16.9650753799944,18.0474255522536,
-18.5650690811547));
#102181=CARTESIAN_POINT('Ctrl Pts',(-16.9454362925661,18.0778454173411,
-18.5627944718622));
#102182=CARTESIAN_POINT('Ctrl Pts',(-16.8845227381142,18.1777284189964,
-18.5553355677207));
#102183=CARTESIAN_POINT('Ctrl Pts',(-16.8464430677305,18.2490522921136,
-18.5500264486163));
#102184=CARTESIAN_POINT('Ctrl Pts',(-16.7350623018389,18.4898890543805,
-18.5325062086297));
#102185=CARTESIAN_POINT('Ctrl Pts',(-16.6798120052927,18.6668568314805,
-18.5203494408362));
#102186=CARTESIAN_POINT('Ctrl Pts',(-16.6444200791822,18.8706503759169,
-18.5076276806556));
#102187=CARTESIAN_POINT('Ctrl Pts',(-16.6409648788929,18.892588076754,-18.506272762166));
#102188=CARTESIAN_POINT('Ctrl Pts',(-16.6366687924886,18.9229676729009,
-18.5044158648713));
#102189=CARTESIAN_POINT('Ctrl Pts',(-16.6355325843793,18.9313657311761,
-18.5039045871614));
#102190=CARTESIAN_POINT('Ctrl Pts',(-16.633667589146,18.9458024219286,-18.5030291118981));
#102191=CARTESIAN_POINT('Ctrl Pts',(-16.6329143483417,18.9518377398332,
-18.5026641456139));
#102192=CARTESIAN_POINT('Ctrl Pts',(-16.6314162863302,18.9642768976401,
-18.5019140171535));
#102193=CARTESIAN_POINT('Ctrl Pts',(-16.6306746865337,18.9706810673731,
-18.5015289603209));
#102194=CARTESIAN_POINT('Ctrl Pts',(-16.6290188354424,18.9855754793064,
-18.5006360198249));
#102195=CARTESIAN_POINT('Ctrl Pts',(-16.6281266721895,18.9940681025113,
-18.5001288370362));
#102196=CARTESIAN_POINT('Ctrl Pts',(-16.6254422588638,19.021200389181,-18.4985145827147));
#102197=CARTESIAN_POINT('Ctrl Pts',(-16.6238458866772,19.0398588554769,
-18.4974136689816));
#102198=CARTESIAN_POINT('Ctrl Pts',(-16.6207015717367,19.0834052108706,
-18.4948641876817));
#102199=CARTESIAN_POINT('Ctrl Pts',(-16.6193453325324,19.1083043921394,
-18.4934215645896));
#102200=CARTESIAN_POINT('Ctrl Pts',(-16.6161236358701,19.1959354658402,
-18.4883909198547));
#102201=CARTESIAN_POINT('Ctrl Pts',(-16.6166075820429,19.2587228882699,
-18.4848714188122));
#102202=CARTESIAN_POINT('Ctrl Pts',(-16.6250763360982,19.4208964994915,
-18.4758936563694));
#102203=CARTESIAN_POINT('Ctrl Pts',(-16.6372896489054,19.5199041061963,
-18.4705265895589));
#102204=CARTESIAN_POINT('Ctrl Pts',(-16.6703757761435,19.688927065847,-18.4611455235353));
#102205=CARTESIAN_POINT('Ctrl Pts',(-16.6879763700105,19.7594024107075,
-18.4571637022484));
#102206=CARTESIAN_POINT('Ctrl Pts',(-16.7224337106618,19.8723309385836,
-18.4504775309333));
#102207=CARTESIAN_POINT('Ctrl Pts',(-16.7371044392647,19.9153898114008,
-18.4478528432147));
#102208=CARTESIAN_POINT('Ctrl Pts',(-16.7558349744706,19.9650623877469,
-18.4447001323656));
#102209=CARTESIAN_POINT('Ctrl Pts',(-16.7585593050228,19.9721708149481,
-18.4442459260524));
#102210=CARTESIAN_POINT('Ctrl Pts',(-16.7629929661602,19.9835551610362,
-18.4435133850684));
#102211=CARTESIAN_POINT('Ctrl Pts',(-16.7646780406065,19.9878405393788,
-18.4432364675873));
#102212=CARTESIAN_POINT('Ctrl Pts',(-16.7676990371587,19.9954503554379,
-18.4427425887856));
#102213=CARTESIAN_POINT('Ctrl Pts',(-16.7690294317274,19.9987769368674,
-18.4425259618986));
#102214=CARTESIAN_POINT('Ctrl Pts',(-16.7718806419747,20.0058540770918,
-18.4420635208414));
#102215=CARTESIAN_POINT('Ctrl Pts',(-16.7734037461362,20.0096035986067,
-18.4418175748332));
#102216=CARTESIAN_POINT('Ctrl Pts',(-16.7775739730624,20.0197858733875,
-18.4411471627926));
#102217=CARTESIAN_POINT('Ctrl Pts',(-16.7802420377899,20.0262099176705,
-18.440721459362));
#102218=CARTESIAN_POINT('Ctrl Pts',(-16.7940581786047,20.0590183658349,
-18.4385337340417));
#102219=CARTESIAN_POINT('Ctrl Pts',(-16.8057086627393,20.0851863359754,
-18.4367436744521));
#102220=CARTESIAN_POINT('Ctrl Pts',(-16.8415930256975,20.1615755179546,
-18.4314010059629));
#102221=CARTESIAN_POINT('Ctrl Pts',(-16.8672833686317,20.2110830646669,
-18.4277867724062));
#102222=CARTESIAN_POINT('Ctrl Pts',(-16.9641148025644,20.380926188453,-18.4149792257097));
#102223=CARTESIAN_POINT('Ctrl Pts',(-17.0451937295155,20.4951959966145,
-18.4056419046629));
#102224=CARTESIAN_POINT('Ctrl Pts',(-17.1956136785661,20.6680671950216,
-18.3908536158708));
#102225=CARTESIAN_POINT('Ctrl Pts',(-17.2584993159252,20.7317164875509,
-18.3852223007828));
#102226=CARTESIAN_POINT('Ctrl Pts',(-17.335455302848,20.8003235761346,-18.3789320111313));
#102227=CARTESIAN_POINT('Ctrl Pts',(-17.3457701912751,20.8093412375359,
-18.3781002816309));
#102228=CARTESIAN_POINT('Ctrl Pts',(-17.3624602970714,20.8236488902854,
-18.3767724235661));
#102229=CARTESIAN_POINT('Ctrl Pts',(-17.3687801563195,20.8290025900825,
-18.3762736669715));
#102230=CARTESIAN_POINT('Ctrl Pts',(-17.3800617019963,20.8384462900963,
-18.375390433832));
#102231=CARTESIAN_POINT('Ctrl Pts',(-17.3850108793157,20.8425510092054,
-18.3750053572364));
#102232=CARTESIAN_POINT('Ctrl Pts',(-17.3953661692853,20.8510600871905,
-18.3742045864678));
#102233=CARTESIAN_POINT('Ctrl Pts',(-17.4007755032213,20.855460417677,-18.3737890584724));
#102234=CARTESIAN_POINT('Ctrl Pts',(-17.4148896843368,20.8668264604222,
-18.3727119634686));
#102235=CARTESIAN_POINT('Ctrl Pts',(-17.4236280616696,20.873750336746,-18.3720520801946));
#102236=CARTESIAN_POINT('Ctrl Pts',(-17.4619075006349,20.9035919582972,
-18.3691910091844));
#102237=CARTESIAN_POINT('Ctrl Pts',(-17.4919991324997,20.9257947287182,
-18.3670181151365));
#102238=CARTESIAN_POINT('Ctrl Pts',(-17.57360358355,20.9827299583572,-18.3613084696117));
#102239=CARTESIAN_POINT('Ctrl Pts',(-17.6260844569564,21.0160127168111,
-18.3578234738029));
#102240=CARTESIAN_POINT('Ctrl Pts',(-17.7615180464885,21.0937673349624,
-18.3491860913571));
#102241=CARTESIAN_POINT('Ctrl Pts',(-17.8461113089125,21.1351071274312,
-18.3441102629351));
#102242=CARTESIAN_POINT('Ctrl Pts',(-18.0471320316314,21.2172543976426,
-18.3322971687134));
#102243=CARTESIAN_POINT('Ctrl Pts',(-18.1649197548056,21.2537880565793,
-18.3255544315244));
#102244=CARTESIAN_POINT('Ctrl Pts',(-18.294420180211,21.2818809072839,-18.3177000941544));
#102245=CARTESIAN_POINT('Ctrl Pts',(-18.3036605879557,21.2838208154799,
-18.3171372495877));
#102246=CARTESIAN_POINT('Ctrl Pts',(-18.3173921952109,21.2866078199623,
-18.3162968628275));
#102247=CARTESIAN_POINT('Ctrl Pts',(-18.321873805411,21.2875023198,-18.3160219571014));
#102248=CARTESIAN_POINT('Ctrl Pts',(-18.329862256082,21.2890698821095,-18.3155307659069));
#102249=CARTESIAN_POINT('Ctrl Pts',(-18.3333679369158,21.2897485900853,
-18.3153148057859));
#102250=CARTESIAN_POINT('Ctrl Pts',(-18.3409196493654,21.2911908063273,
-18.3148487135619));
#102251=CARTESIAN_POINT('Ctrl Pts',(-18.3449661373781,21.2919513703712,
-18.3145984231655));
#102252=CARTESIAN_POINT('Ctrl Pts',(-18.3561680328796,21.2940230252584,
-18.3139040976406));
#102253=CARTESIAN_POINT('Ctrl Pts',(-18.3633279397275,21.2953090316292,
-18.3134586750977));
#102254=CARTESIAN_POINT('Ctrl Pts',(-18.401803121093,21.3020151268502,-18.3110568826375));
#102255=CARTESIAN_POINT('Ctrl Pts',(-18.4332290461028,21.3067661149977,
-18.309065955719));
#102256=CARTESIAN_POINT('Ctrl Pts',(-18.6266527132522,21.3315682526454,
-18.2966817144529));
#102257=CARTESIAN_POINT('Ctrl Pts',(-18.7904105055977,21.3335340649681,
-18.2856881651653));
#102258=CARTESIAN_POINT('Ctrl Pts',(-19.0691176224929,21.3045780093424,
-18.2673840949449));
#102259=CARTESIAN_POINT('Ctrl Pts',(-19.184281020735,21.2828657153222,-18.2599322079371));
#102260=CARTESIAN_POINT('Ctrl Pts',(-19.3108537418502,21.2479420728577,
-18.2519148693099));
#102261=CARTESIAN_POINT('Ctrl Pts',(-19.3245918804956,21.2440013512247,
-18.2510467591403));
#102262=CARTESIAN_POINT('Ctrl Pts',(-19.3463926963135,21.2375082469543,
-18.249672278985));
#102263=CARTESIAN_POINT('Ctrl Pts',(-19.3544816211667,21.2350462076016,
-18.249162979794));
#102264=CARTESIAN_POINT('Ctrl Pts',(-19.3687213290974,21.2306186582975,
-18.2482675567575));
#102265=CARTESIAN_POINT('Ctrl Pts',(-19.3748782359761,21.2286733577662,
-18.2478807765782));
#102266=CARTESIAN_POINT('Ctrl Pts',(-19.3875939364863,21.2245917028674,
-18.2470827163397));
#102267=CARTESIAN_POINT('Ctrl Pts',(-19.3941513888815,21.2224513976623,
-18.2466715715529));
#102268=CARTESIAN_POINT('Ctrl Pts',(-19.4109558812591,21.2168755037443,
-18.2456189455179));
#102269=CARTESIAN_POINT('Ctrl Pts',(-19.4211873656841,21.2133934010812,
-18.2449790050895));
#102270=CARTESIAN_POINT('Ctrl Pts',(-19.4631591849632,21.1987494536888,
-18.2423573175786));
#102271=CARTESIAN_POINT('Ctrl Pts',(-19.4946589458198,21.1869097048001,
-18.2403980965002));
#102272=CARTESIAN_POINT('Ctrl Pts',(-19.5758782853012,21.1541516269173,
-18.2353573405987));
#102273=CARTESIAN_POINT('Ctrl Pts',(-19.6251053130139,21.1320750178919,
-18.232313460381));
#102274=CARTESIAN_POINT('Ctrl Pts',(-19.7875131334145,21.0516528946919,
-18.2222267901521));
#102275=CARTESIAN_POINT('Ctrl Pts',(-19.8962588136807,20.9849920601618,
-18.2154131056184));
#102276=CARTESIAN_POINT('Ctrl Pts',(-20.0802520402526,20.8479849206862,
-18.2028688011266));
#102277=CARTESIAN_POINT('Ctrl Pts',(-20.1576161874521,20.781167365725,-18.1972001957628));
#102278=CARTESIAN_POINT('Ctrl Pts',(-20.2367056090523,20.7021937393487,
-18.1905785829377));
#102279=CARTESIAN_POINT('Ctrl Pts',(-20.2435159618116,20.6952993191145,
-18.1900010840718));
#102280=CARTESIAN_POINT('Ctrl Pts',(-20.253501809508,20.6850504006879,-18.1891429902576));
#102281=CARTESIAN_POINT('Ctrl Pts',(-20.2567141574148,20.6817317657371,
-18.1888651959223));
#102282=CARTESIAN_POINT('Ctrl Pts',(-20.2623940489886,20.6758253876297,
-18.1883708351796));
#102283=CARTESIAN_POINT('Ctrl Pts',(-20.2648659238849,20.6732418774289,
-18.1881546104882));
#102284=CARTESIAN_POINT('Ctrl Pts',(-20.2701482855966,20.6676928767169,
-18.1876902036748));
#102285=CARTESIAN_POINT('Ctrl Pts',(-20.272956694062,20.6647255537303,-18.1874418751137));
#102286=CARTESIAN_POINT('Ctrl Pts',(-20.2787023602443,20.6586194588903,
-18.1869309311276));
#102287=CARTESIAN_POINT('Ctrl Pts',(-20.281638680851,20.6554798345072,-18.1866682475573));
#102288=CARTESIAN_POINT('Ctrl Pts',(-20.2950923992441,20.6410065001642,
-18.1854575478593));
#102289=CARTESIAN_POINT('Ctrl Pts',(-20.3054946772955,20.6295670646149,
-18.1845013204067));
#102290=CARTESIAN_POINT('Ctrl Pts',(-20.373802653567,20.5527750441598,-18.1780928773938));
#102291=CARTESIAN_POINT('Ctrl Pts',(-20.4277374315298,20.4840135069281,
-18.1724082714805));
#102292=CARTESIAN_POINT('Ctrl Pts',(-20.5185485974922,20.3522138435245,
-18.1618726270031));
#102293=CARTESIAN_POINT('Ctrl Pts',(-20.5567134720684,20.290211972345,-18.1570467852984));
#102294=CARTESIAN_POINT('Ctrl Pts',(-20.5938938829306,20.2221905888911,
-18.1519487435824));
#102295=CARTESIAN_POINT('Ctrl Pts',(-20.5961630741471,20.2180056347125,
-18.1516358473825));
#102296=CARTESIAN_POINT('Ctrl Pts',(-20.6621519663309,20.0953198686994,
-18.1424854513605));
#102297=CARTESIAN_POINT('Ctrl Pts',(-20.7144538820208,19.9710037717547,
-18.1338552316719));
#102298=CARTESIAN_POINT('Ctrl Pts',(-20.7593062374906,19.8274998292925,
-18.1246739477026));
#102299=CARTESIAN_POINT('Ctrl Pts',(-20.7638398849016,19.8124045708868,
-18.123717027009));
#102300=CARTESIAN_POINT('Ctrl Pts',(-20.7704399625781,19.7895036156674,
-18.1222783558662));
#102301=CARTESIAN_POINT('Ctrl Pts',(-20.7726309376648,19.7817346645665,
-18.1217925574626));
#102302=CARTESIAN_POINT('Ctrl Pts',(-20.7764755274864,19.7677975362387,
-18.1209250381826));
#102303=CARTESIAN_POINT('Ctrl Pts',(-20.7781457594234,19.7616340820893,
-18.1205427810745));
#102304=CARTESIAN_POINT('Ctrl Pts',(-20.78162868502,19.7485471941944,-18.119734034827));
#102305=CARTESIAN_POINT('Ctrl Pts',(-20.7834342132145,19.7416219231616,
-18.1193077820769));
#102306=CARTESIAN_POINT('Ctrl Pts',(-20.7870375877092,19.7275080528404,
-18.1184424999487));
#102307=CARTESIAN_POINT('Ctrl Pts',(-20.7888328801429,19.7203189000964,
-18.1180035578064));
#102308=CARTESIAN_POINT('Ctrl Pts',(-20.7932123060319,19.7023815980453,
-18.1169127792003));
#102309=CARTESIAN_POINT('Ctrl Pts',(-20.7957500888887,19.6916222779489,
-18.1162624274975));
#102310=CARTESIAN_POINT('Ctrl Pts',(-20.8334344277754,19.5260604299048,
-18.1063132200247));
#102311=CARTESIAN_POINT('Ctrl Pts',(-20.8511450351187,19.3678091395082,
-18.0976370754808));
#102312=CARTESIAN_POINT('Ctrl Pts',(-20.8509991056215,19.209054030408,-18.0890148055994));
#102313=CARTESIAN_POINT('Ctrl Pts',(-20.8509991057282,19.2090541464559,
-18.0890148119022));
#102314=CARTESIAN_POINT('Ctrl Pts',(-20.8508677556262,19.0661512803534,
-18.0812535052745));
#102315=CARTESIAN_POINT('Ctrl Pts',(-20.8362673125345,18.9236435276234,
-18.0735576995762));
#102316=CARTESIAN_POINT('Ctrl Pts',(-20.8054605704913,18.7741529475324,
-18.0645866360258));
#102317=CARTESIAN_POINT('Ctrl Pts',(-20.8034247687687,18.7646085115214,
-18.0640097962226));
#102318=CARTESIAN_POINT('Ctrl Pts',(-20.8001177070468,18.7496130180313,
-18.0630966111073));
#102319=CARTESIAN_POINT('Ctrl Pts',(-20.7988906685246,18.7441522175532,
-18.0627626188202));
#102320=CARTESIAN_POINT('Ctrl Pts',(-20.7965252968809,18.7338171694132,
-18.0621276602403));
#102321=CARTESIAN_POINT('Ctrl Pts',(-20.7953913008448,18.7289419560779,
-18.0618269359283));
#102322=CARTESIAN_POINT('Ctrl Pts',(-20.7934049810816,18.7205376622443,
-18.0613063720389));
#102323=CARTESIAN_POINT('Ctrl Pts',(-20.792560840268,18.717006631999,-18.0610870021718));
#102324=CARTESIAN_POINT('Ctrl Pts',(-20.7909046571635,18.7101568059559,
-18.060660145096));
#102325=CARTESIAN_POINT('Ctrl Pts',(-20.7900936622065,18.7068377983904,
-18.0604527244233));
#102326=CARTESIAN_POINT('Ctrl Pts',(-20.7878798168748,18.6978717951775,
-18.0598908229163));
#102327=CARTESIAN_POINT('Ctrl Pts',(-20.7864617259332,18.6922286452664,
-18.059535476532));
#102328=CARTESIAN_POINT('Ctrl Pts',(-20.7810875036896,18.6712094602303,
-18.0582057915177));
#102329=CARTESIAN_POINT('Ctrl Pts',(-20.7769818152394,18.6558726787763,
-18.0572233519935));
#102330=CARTESIAN_POINT('Ctrl Pts',(-20.7580005331028,18.5880323254332,
-18.0528276743546));
#102331=CARTESIAN_POINT('Ctrl Pts',(-20.7412781925629,18.5360963365021,
-18.0493294498771));
#102332=CARTESIAN_POINT('Ctrl Pts',(-20.7225806765445,18.484889889291,-18.0457834329553));
#102333=CARTESIAN_POINT('Origin',(-18.734,19.211,0.));
#102334=CARTESIAN_POINT('',(-20.7225806138883,18.484889717696,-17.2426990599955));
#102335=CARTESIAN_POINT('',(-20.7225806135343,18.4848897167264,-17.4677765237272));
#102336=CARTESIAN_POINT('',(-20.7225806137986,18.4848897174502,0.));
#102337=CARTESIAN_POINT('Ctrl Pts',(-20.7225806135343,18.4848897167264,
-17.4677765237272));
#102338=CARTESIAN_POINT('Ctrl Pts',(-20.7401855017382,18.5331037968631,
-17.4710694629831));
#102339=CARTESIAN_POINT('Ctrl Pts',(-20.7560325936953,18.5819462166473,
-17.4743159902952));
#102340=CARTESIAN_POINT('Ctrl Pts',(-20.7795153171967,18.6644279559498,
-17.479647141129));
#102341=CARTESIAN_POINT('Ctrl Pts',(-20.7881324561808,18.6977612804346,
-17.4817614807328));
#102342=CARTESIAN_POINT('Ctrl Pts',(-20.798385541561,18.7418321682609,-17.4845061478134));
#102343=CARTESIAN_POINT('Ctrl Pts',(-20.8007569905954,18.7523915971316,
-17.4851599905889));
#102344=CARTESIAN_POINT('Ctrl Pts',(-20.8045078945201,18.7697136045771,
-17.4862265075556));
#102345=CARTESIAN_POINT('Ctrl Pts',(-20.8059354157485,18.7764654688328,
-17.4866407168297));
#102346=CARTESIAN_POINT('Ctrl Pts',(-20.8086343584051,18.78954661849,-17.4874403466462));
#102347=CARTESIAN_POINT('Ctrl Pts',(-20.8099098928635,18.7958749682356,
-17.4878258947998));
#102348=CARTESIAN_POINT('Ctrl Pts',(-20.8127876279131,18.8104973732348,
-17.488713811454));
#102349=CARTESIAN_POINT('Ctrl Pts',(-20.814369179777,18.8187954169063,-17.4892155163142));
#102350=CARTESIAN_POINT('Ctrl Pts',(-20.8184877298123,18.8411305981548,
-17.4905602003735));
#102351=CARTESIAN_POINT('Ctrl Pts',(-20.8209326213357,18.8551844312056,
-17.4914002514707));
#102352=CARTESIAN_POINT('Ctrl Pts',(-20.8418093122528,18.9828153677844,
-17.498976914763));
#102353=CARTESIAN_POINT('Ctrl Pts',(-20.8510962906784,19.0977007821835,
-17.5054071166955));
#102354=CARTESIAN_POINT('Ctrl Pts',(-20.8508421937833,19.3990360594247,
-17.5219135397002));
#102355=CARTESIAN_POINT('Ctrl Pts',(-20.8261075478748,19.5844189879619,
-17.5316811244396));
#102356=CARTESIAN_POINT('Ctrl Pts',(-20.7737437540893,19.7778655756826,
-17.5434580816054));
#102357=CARTESIAN_POINT('Ctrl Pts',(-20.7698906310782,19.7915518728401,
-17.5443004711881));
#102358=CARTESIAN_POINT('Ctrl Pts',(-20.7643392702007,19.8105351281857,
-17.5454830104063));
#102359=CARTESIAN_POINT('Ctrl Pts',(-20.7627574776275,19.8158661152896,
-17.5458166554832));
#102360=CARTESIAN_POINT('Ctrl Pts',(-20.7601843571699,19.8244144477096,
-17.546354256482));
#102361=CARTESIAN_POINT('Ctrl Pts',(-20.7592063131648,19.8276358103852,
-17.5465574398533));
#102362=CARTESIAN_POINT('Ctrl Pts',(-20.7571469224101,19.8343610324556,
-17.5469828914886));
#102363=CARTESIAN_POINT('Ctrl Pts',(-20.7560641553507,19.8378644170424,
-17.5472052452409));
#102364=CARTESIAN_POINT('Ctrl Pts',(-20.753422272186,19.8463343881325,-17.5477445402991));
#102365=CARTESIAN_POINT('Ctrl Pts',(-20.7518539338272,19.8512980544694,
-17.5480620177548));
#102366=CARTESIAN_POINT('Ctrl Pts',(-20.746300568609,19.8686509684515,-17.5491768136078));
#102367=CARTESIAN_POINT('Ctrl Pts',(-20.7422197101637,19.8810089186436,
-17.5499794781113));
#102368=CARTESIAN_POINT('Ctrl Pts',(-20.7174287549397,19.9538209592796,
-17.554757362591));
#102369=CARTESIAN_POINT('Ctrl Pts',(-20.6941056009685,20.0133447400581,
-17.5588615753347));
#102370=CARTESIAN_POINT('Ctrl Pts',(-20.5919077580978,20.2429950445904,
-17.5752528778096));
#102371=CARTESIAN_POINT('Ctrl Pts',(-20.4932538776527,20.403426203793,-17.5878515549434));
#102372=CARTESIAN_POINT('Ctrl Pts',(-20.339345532912,20.5921931517566,-17.6032548905438));
#102373=CARTESIAN_POINT('Ctrl Pts',(-20.3022242623432,20.6342014585516,
-17.6067354325915));
#102374=CARTESIAN_POINT('Ctrl Pts',(-20.2551575013988,20.6833836584273,
-17.6108793456923));
#102375=CARTESIAN_POINT('Ctrl Pts',(-20.2467641375125,20.6920058930676,
-17.6116085810263));
#102376=CARTESIAN_POINT('Ctrl Pts',(-20.2327633285163,20.7061452605599,
-17.6128091802791));
#102377=CARTESIAN_POINT('Ctrl Pts',(-20.2271979156031,20.7117034525592,
-17.6132823734987));
#102378=CARTESIAN_POINT('Ctrl Pts',(-20.2170712362349,20.7217048858146,
-17.6141361456632));
#102379=CARTESIAN_POINT('Ctrl Pts',(-20.2125206755465,20.7261587894095,
-17.6145171931039));
#102380=CARTESIAN_POINT('Ctrl Pts',(-20.2027146364378,20.7356702968274,
-17.6153327865034));
#102381=CARTESIAN_POINT('Ctrl Pts',(-20.1974529644605,20.7407214191377,
-17.6157670469204));
#102382=CARTESIAN_POINT('Ctrl Pts',(-20.1830322554327,20.7544225698834,
-17.6169481756598));
#102383=CARTESIAN_POINT('Ctrl Pts',(-20.1738218512727,20.7630182838601,
-17.6176926990876));
#102384=CARTESIAN_POINT('Ctrl Pts',(-20.1246865380443,20.8080604985663,
-17.6216137907165));
#102385=CARTESIAN_POINT('Ctrl Pts',(-20.0834512976085,20.8430518380806,
-17.6247285140547));
#102386=CARTESIAN_POINT('Ctrl Pts',(-19.8904550279948,20.994502633775,-17.6386249558782));
#102387=CARTESIAN_POINT('Ctrl Pts',(-19.7246997223292,21.0916324078305,
-17.648649131046));
#102388=CARTESIAN_POINT('Ctrl Pts',(-19.532889788244,21.1715452891823,-17.6602001879931));
#102389=CARTESIAN_POINT('Ctrl Pts',(-19.5175438116647,21.1777287052002,
-17.6611246906026));
#102390=CARTESIAN_POINT('Ctrl Pts',(-19.4525633609,21.2030303001758,-17.6650468672106));
#102391=CARTESIAN_POINT('Ctrl Pts',(-19.4022941167739,21.2204526575283,
-17.6680992391007));
#102392=CARTESIAN_POINT('Ctrl Pts',(-19.3430951510089,21.2385028907138,
-17.6717720244273));
#102393=CARTESIAN_POINT('Ctrl Pts',(-19.3347477946261,21.2409918611138,
-17.6722916909952));
#102394=CARTESIAN_POINT('Ctrl Pts',(-19.3220833337508,21.2446831300285,
-17.6730831509535));
#102395=CARTESIAN_POINT('Ctrl Pts',(-19.3177772636195,21.245923385887,-17.6733527857104));
#102396=CARTESIAN_POINT('Ctrl Pts',(-19.3100395985306,21.2481254457913,
-17.6738383000373));
#102397=CARTESIAN_POINT('Ctrl Pts',(-19.3066094866584,21.2490922639705,
-17.6740538842183));
#102398=CARTESIAN_POINT('Ctrl Pts',(-19.2991494074299,21.251174657215,-17.6745235372396));
#102399=CARTESIAN_POINT('Ctrl Pts',(-19.2951186240095,21.2522869405726,
-17.6747777879111));
#102400=CARTESIAN_POINT('Ctrl Pts',(-19.2837833323716,21.2553787717146,
-17.6754941120813));
#102401=CARTESIAN_POINT('Ctrl Pts',(-19.2764715518758,21.2573310793282,
-17.6759577176318));
#102402=CARTESIAN_POINT('Ctrl Pts',(-19.2326173819694,21.2687889621607,
-17.678746880659));
#102403=CARTESIAN_POINT('Ctrl Pts',(-19.1958388841269,21.2773540702253,
-17.6811215430674));
#102404=CARTESIAN_POINT('Ctrl Pts',(-19.0738711903075,21.3023396898997,
-17.6890698828279));
#102405=CARTESIAN_POINT('Ctrl Pts',(-18.9879041063387,21.314507765477,-17.6947856458968));
#102406=CARTESIAN_POINT('Ctrl Pts',(-18.7261753247924,21.3352736700453,
-17.7121323654626));
#102407=CARTESIAN_POINT('Ctrl Pts',(-18.5498247968382,21.3272946240507,
-17.7236767744086));
#102408=CARTESIAN_POINT('Ctrl Pts',(-18.3538349909117,21.293712395024,-17.7359157952053));
#102409=CARTESIAN_POINT('Ctrl Pts',(-18.3312645955787,21.289465927971,-17.7373176563944));
#102410=CARTESIAN_POINT('Ctrl Pts',(-18.2994198014168,21.2829363154545,
-17.7392854628916));
#102411=CARTESIAN_POINT('Ctrl Pts',(-18.2900855071934,21.2809565145285,
-17.7398610319646));
#102412=CARTESIAN_POINT('Ctrl Pts',(-18.2749371285508,21.2776363669525,
-17.7407931868183));
#102413=CARTESIAN_POINT('Ctrl Pts',(-18.2691148405509,21.276334448173,-17.741150998533));
#102414=CARTESIAN_POINT('Ctrl Pts',(-18.2569362181612,21.2735570843908,
-17.7418985026749));
#102415=CARTESIAN_POINT('Ctrl Pts',(-18.2505810368542,21.2720768267715,
-17.7422880361825));
#102416=CARTESIAN_POINT('Ctrl Pts',(-18.2354734744866,21.2684842324869,
-17.7432128060565));
#102417=CARTESIAN_POINT('Ctrl Pts',(-18.2267274796152,21.2663453864129,
-17.7437471833));
#102418=CARTESIAN_POINT('Ctrl Pts',(-18.1972848267411,21.2589457606144,
-17.7455429939267));
#102419=CARTESIAN_POINT('Ctrl Pts',(-18.1766537735633,21.2534275381563,
-17.746796116402));
#102420=CARTESIAN_POINT('Ctrl Pts',(-18.0646429720959,21.221644134476,-17.7535762391585));
#102421=CARTESIAN_POINT('Ctrl Pts',(-17.9750234795633,21.1895566352275,
-17.7589089307374));
#102422=CARTESIAN_POINT('Ctrl Pts',(-17.7316856130007,21.0834532436264,
-17.7735136302517));
#102423=CARTESIAN_POINT('Ctrl Pts',(-17.5843250381929,20.9967633772086,
-17.7824762307702));
#102424=CARTESIAN_POINT('Ctrl Pts',(-17.4194444096351,20.8708228937859,
-17.7943223132381));
#102425=CARTESIAN_POINT('Ctrl Pts',(-17.3905292247996,20.8475067486092,
-17.7964791248145));
#102426=CARTESIAN_POINT('Ctrl Pts',(-17.3567880977732,20.8188021307609,
-17.7991126703789));
#102427=CARTESIAN_POINT('Ctrl Pts',(-17.3513556187075,20.8141328163614,
-17.7995404077042));
#102428=CARTESIAN_POINT('Ctrl Pts',(-17.342535023044,20.8064731707622,-17.8002412142003));
#102429=CARTESIAN_POINT('Ctrl Pts',(-17.3391325480752,20.8034993599396,
-17.800513088652));
#102430=CARTESIAN_POINT('Ctrl Pts',(-17.3330617886125,20.7981590493674,
-17.8010009970408));
#102431=CARTESIAN_POINT('Ctrl Pts',(-17.3303899401623,20.795796680892,-17.8012167228393));
#102432=CARTESIAN_POINT('Ctrl Pts',(-17.3246195900884,20.7906686706827,
-17.8016847806611));
#102433=CARTESIAN_POINT('Ctrl Pts',(-17.3215232961562,20.7879006973786,
-17.801937284191));
#102434=CARTESIAN_POINT('Ctrl Pts',(-17.3129044808975,20.7801500410381,
-17.8026438769515));
#102435=CARTESIAN_POINT('Ctrl Pts',(-17.3074001082275,20.7751473941808,
-17.8030994334585));
#102436=CARTESIAN_POINT('Ctrl Pts',(-17.2757262840235,20.746054383076,-17.8057451865685));
#102437=CARTESIAN_POINT('Ctrl Pts',(-17.2501425757728,20.7213380379271,
-17.8079789114837));
#102438=CARTESIAN_POINT('Ctrl Pts',(-17.1701688941047,20.6400818718344,
-17.8152436471109));
#102439=CARTESIAN_POINT('Ctrl Pts',(-17.1182960689422,20.5811612570308,
-17.8203928897734));
#102440=CARTESIAN_POINT('Ctrl Pts',(-16.9535227908271,20.3715988317451,
-17.8379884213599));
#102441=CARTESIAN_POINT('Ctrl Pts',(-16.8574389357575,20.2088156622849,
-17.8503967891509));
#102442=CARTESIAN_POINT('Ctrl Pts',(-16.7756319364519,20.0153384689312,
-17.8633116409322));
#102443=CARTESIAN_POINT('Ctrl Pts',(-16.767439216009,19.9950947543902,-17.8646436958221));
#102444=CARTESIAN_POINT('Ctrl Pts',(-16.7565247311852,19.9668778953813,
-17.866474504849));
#102445=CARTESIAN_POINT('Ctrl Pts',(-16.7535353304409,19.959010379158,-17.8669822213399));
#102446=CARTESIAN_POINT('Ctrl Pts',(-16.7484719090493,19.945441287623,-17.8678532078645));
#102447=CARTESIAN_POINT('Ctrl Pts',(-16.7463753511042,19.9397482838492,
-17.8682172289767));
#102448=CARTESIAN_POINT('Ctrl Pts',(-16.7420986081804,19.9279794367077,
-17.8689668815873));
#102449=CARTESIAN_POINT('Ctrl Pts',(-16.7399216800821,19.9219024707035,
-17.8693524012691));
#102450=CARTESIAN_POINT('Ctrl Pts',(-16.7349121175787,19.9077140414799,
-17.8702488977921));
#102451=CARTESIAN_POINT('Ctrl Pts',(-16.7321009872935,19.899595064957,-17.8707591561239));
#102452=CARTESIAN_POINT('Ctrl Pts',(-16.7232285355061,19.8734564550765,
-17.872393289621));
#102453=CARTESIAN_POINT('Ctrl Pts',(-16.717360383947,19.8553718888468,-17.8735107878467));
#102454=CARTESIAN_POINT('Ctrl Pts',(-16.6890932315124,19.7640868483366,
-17.8790893020267));
#102455=CARTESIAN_POINT('Ctrl Pts',(-16.6704313017467,19.6897846862073,
-17.8834272040591));
#102456=CARTESIAN_POINT('Ctrl Pts',(-16.6348812019892,19.5067474962954,
-17.8937893867801));
#102457=CARTESIAN_POINT('Ctrl Pts',(-16.6223602186109,19.3973989326201,
-17.8997042896731));
#102458=CARTESIAN_POINT('Ctrl Pts',(-16.6158407657569,19.21726838309,-17.9095210497298));
#102459=CARTESIAN_POINT('Ctrl Pts',(-16.6168022693298,19.1468873021952,
-17.9133779394741));
#102460=CARTESIAN_POINT('Ctrl Pts',(-16.6243087937617,19.0288080833941,
-17.9200628991658));
#102461=CARTESIAN_POINT('Ctrl Pts',(-16.6289792851901,18.9810480340628,
-17.9228265846165));
#102462=CARTESIAN_POINT('Ctrl Pts',(-16.6362812414009,18.9258249278941,
-17.9261338217255));
#102463=CARTESIAN_POINT('Ctrl Pts',(-16.6373370215447,18.9181635907677,
-17.9265951617907));
#102464=CARTESIAN_POINT('Ctrl Pts',(-16.6390934126413,18.9059148907293,
-17.9273370070947));
#102465=CARTESIAN_POINT('Ctrl Pts',(-16.6397671807793,18.9013236663577,
-17.9276160371743));
#102466=CARTESIAN_POINT('Ctrl Pts',(-16.6409885716106,18.8931871149466,
-17.9281122978151));
#102467=CARTESIAN_POINT('Ctrl Pts',(-16.6415301168857,18.8896409214478,
-17.9283291822336));
#102468=CARTESIAN_POINT('Ctrl Pts',(-16.6426986196792,18.8821174250364,
-17.9287906053366));
#102469=CARTESIAN_POINT('Ctrl Pts',(-16.6433279011421,18.8781405914226,
-17.9290352678897));
#102470=CARTESIAN_POINT('Ctrl Pts',(-16.6450604254318,18.8673904112795,
-17.9296986501418));
#102471=CARTESIAN_POINT('Ctrl Pts',(-16.6461852541719,18.8606206630246,
-17.9301185645419));
#102472=CARTESIAN_POINT('Ctrl Pts',(-16.6519790006109,18.8267699403666,
-17.9322286700516));
#102473=CARTESIAN_POINT('Ctrl Pts',(-16.6571417652368,18.799777570755,-17.9339446224644));
#102474=CARTESIAN_POINT('Ctrl Pts',(-16.6736716341648,18.7216314860609,
-17.9389949988822));
#102475=CARTESIAN_POINT('Ctrl Pts',(-16.6864139312297,18.6707916448975,
-17.9423839237506));
#102476=CARTESIAN_POINT('Ctrl Pts',(-16.7400427017259,18.4861647181204,
-17.9549557968131));
#102477=CARTESIAN_POINT('Ctrl Pts',(-16.7922768025696,18.3560336899456,
-17.9643088319393));
#102478=CARTESIAN_POINT('Ctrl Pts',(-16.9003234586108,18.1488746997371,
-17.9794199513256));
#102479=CARTESIAN_POINT('Ctrl Pts',(-16.9491609184168,18.0687069461899,
-17.985337714743));
#102480=CARTESIAN_POINT('Ctrl Pts',(-17.0111142392699,17.980738045826,-17.9919033924047));
#102481=CARTESIAN_POINT('Ctrl Pts',(-17.0191787029997,17.9695219478511,
-17.9927421000779));
#102482=CARTESIAN_POINT('Ctrl Pts',(-17.0322729491753,17.9516814550668,
-17.9940789146032));
#102483=CARTESIAN_POINT('Ctrl Pts',(-17.0372328847845,17.9450065114993,
-17.9945797061127));
#102484=CARTESIAN_POINT('Ctrl Pts',(-17.046100363026,17.9332186329614,-17.9954652800468));
#102485=CARTESIAN_POINT('Ctrl Pts',(-17.0499921053631,17.9280939946098,
-17.9958506733455));
#102486=CARTESIAN_POINT('Ctrl Pts',(-17.0581403101354,17.9174654204216,
-17.9966508600066));
#102487=CARTESIAN_POINT('Ctrl Pts',(-17.0624006673761,17.9119645572096,
-17.9970654933702));
#102488=CARTESIAN_POINT('Ctrl Pts',(-17.07351521257,17.8977589637143,-17.9981376061424));
#102489=CARTESIAN_POINT('Ctrl Pts',(-17.080410808674,17.8890867872441,-17.998793431286));
#102490=CARTESIAN_POINT('Ctrl Pts',(-17.1104638535129,17.8518940291715,
-18.0016123670032));
#102491=CARTESIAN_POINT('Ctrl Pts',(-17.1342942784982,17.8239237572226,
-18.0037482259425));
#102492=CARTESIAN_POINT('Ctrl Pts',(-17.1993307128797,17.7514960808774,
-18.0093369078352));
#102493=CARTESIAN_POINT('Ctrl Pts',(-17.2417390417962,17.7081628290951,
-18.0127407925299));
#102494=CARTESIAN_POINT('Ctrl Pts',(-17.4051227625998,17.5549616247987,
-18.0251420618489));
#102495=CARTESIAN_POINT('Ctrl Pts',(-17.5368178052085,17.4573962770316,
-18.0337549347408));
#102496=CARTESIAN_POINT('Ctrl Pts',(-17.7277458751237,17.3475673864056,
-18.0461063587303));
#102497=CARTESIAN_POINT('Ctrl Pts',(-17.7782018912341,17.3211912185194,
-18.0493640336671));
#102498=CARTESIAN_POINT('Ctrl Pts',(-17.8376620574325,17.2930986114799,
-18.0532655104877));
#102499=CARTESIAN_POINT('Ctrl Pts',(-17.8456935988078,17.2893654939656,
-18.0537937880132));
#102500=CARTESIAN_POINT('Ctrl Pts',(-17.8578521232322,17.2838066363091,
-18.0545958068095));
#102501=CARTESIAN_POINT('Ctrl Pts',(-17.8619620223047,17.2819434617903,
-18.054867302408));
#102502=CARTESIAN_POINT('Ctrl Pts',(-17.8693303735596,17.2786314653362,
-18.0553548038713));
#102503=CARTESIAN_POINT('Ctrl Pts',(-17.8725865564176,17.2771777238878,
-18.0555705037516));
#102504=CARTESIAN_POINT('Ctrl Pts',(-17.8796473691379,17.2740467558734,
-18.0560388225161));
#102505=CARTESIAN_POINT('Ctrl Pts',(-17.8834532197337,17.2723725314838,
-18.056291614618));
#102506=CARTESIAN_POINT('Ctrl Pts',(-17.8941008105343,17.2677259595913,
-18.0569998117208));
#102507=CARTESIAN_POINT('Ctrl Pts',(-17.9009532867877,17.264778580328,-18.05745669459));
#102508=CARTESIAN_POINT('Ctrl Pts',(-17.9408923290698,17.2478496155883,
-18.06012541439));
#102509=CARTESIAN_POINT('Ctrl Pts',(-17.9743127827382,17.2346765987319,
-18.0623816493635));
#102510=CARTESIAN_POINT('Ctrl Pts',(-18.0829466238835,17.1950199450604,
-18.0697528868596));
#102511=CARTESIAN_POINT('Ctrl Pts',(-18.1593235042396,17.1719337179707,
-18.0749897188038));
#102512=CARTESIAN_POINT('Ctrl Pts',(-18.4177801794577,17.1094875973268,
-18.0925434068086));
#102513=CARTESIAN_POINT('Ctrl Pts',(-18.6037654070718,17.0898172640501,
-18.1048130633488));
#102514=CARTESIAN_POINT('Ctrl Pts',(-18.8119854703271,17.0953220357282,
-18.1176218690414));
#102515=CARTESIAN_POINT('Ctrl Pts',(-18.8340129485203,17.0962488444504,
-18.1189668128272));
#102516=CARTESIAN_POINT('Ctrl Pts',(-18.8644577863475,17.0980065888805,
-18.12081234421));
#102517=CARTESIAN_POINT('Ctrl Pts',(-18.8728900698285,17.098544097219,-18.1213220830863));
#102518=CARTESIAN_POINT('Ctrl Pts',(-18.8873796929115,17.0995548597065,
-18.1221956180186));
#102519=CARTESIAN_POINT('Ctrl Pts',(-18.8934385800864,17.1000037302157,
-18.1225601751643));
#102520=CARTESIAN_POINT('Ctrl Pts',(-18.9059260984624,17.1009829328824,
-18.123310093654));
#102521=CARTESIAN_POINT('Ctrl Pts',(-18.9123544122758,17.1015165770021,
-18.1236953468707));
#102522=CARTESIAN_POINT('Ctrl Pts',(-18.9273092110382,17.1028268926181,
-18.1245898067636));
#102523=CARTESIAN_POINT('Ctrl Pts',(-18.9358336618118,17.1036259283162,
-18.1250983050296));
#102524=CARTESIAN_POINT('Ctrl Pts',(-18.9631072862941,17.1063494168758,
-18.1267210427773));
#102525=CARTESIAN_POINT('Ctrl Pts',(-18.98183602836,17.1084725774156,-18.1278290314348));
#102526=CARTESIAN_POINT('Ctrl Pts',(-19.075264635266,17.1203297704018,-18.1333277643457));
#102527=CARTESIAN_POINT('Ctrl Pts',(-19.1494399374305,17.1337963651649,
-18.1375994757886));
#102528=CARTESIAN_POINT('Ctrl Pts',(-19.388582866453,17.1905395078047,-18.1512689195985));
#102529=CARTESIAN_POINT('Ctrl Pts',(-19.5490461983368,17.2497676839973,
-18.1602348803489));
#102530=CARTESIAN_POINT('Ctrl Pts',(-19.7075115497828,17.3311001337633,
-18.170209306771));
#102531=CARTESIAN_POINT('Ctrl Pts',(-19.714340044477,17.33465204729,-18.1706415377684));
#102532=CARTESIAN_POINT('Ctrl Pts',(-19.7666465489977,17.3622233010299,
-18.1739721943461));
#102533=CARTESIAN_POINT('Ctrl Pts',(-19.8112511998049,17.3878535145652,
-18.1769274241472));
#102534=CARTESIAN_POINT('Ctrl Pts',(-19.8621406753092,17.419614786967,-18.1804878549526));
#102535=CARTESIAN_POINT('Ctrl Pts',(-19.8693791899731,17.4241937838352,
-18.1809988849493));
#102536=CARTESIAN_POINT('Ctrl Pts',(-19.8802944931801,17.4311917790733,
-18.1817767893069));
#102537=CARTESIAN_POINT('Ctrl Pts',(-19.8839919529383,17.4335785880251,
-18.182041575074));
#102538=CARTESIAN_POINT('Ctrl Pts',(-19.8905259528545,17.4378253819979,
-18.1825118108566));
#102539=CARTESIAN_POINT('Ctrl Pts',(-19.8933654925071,17.4396806724508,
-18.1827169462355));
#102540=CARTESIAN_POINT('Ctrl Pts',(-19.8962227854308,17.4415573765363,
-18.1829241589128));
#102541=CARTESIAN_POINT('Ctrl Pts',(-19.8962449713584,17.4415719491156,
-18.1829257678984));
#102542=CARTESIAN_POINT('Ctrl Pts',(-19.8962888781377,17.4416007899762,
-18.1829289522362));
#102543=CARTESIAN_POINT('Ctrl Pts',(-19.8963105991032,17.4416150583076,
-18.1829305275947));
#102544=CARTESIAN_POINT('Ctrl Pts',(-19.8963536046105,17.4416433094208,
-18.1829336467506));
#102545=CARTESIAN_POINT('Ctrl Pts',(-19.8963748891621,17.4416572921861,
-18.1829351905469));
#102546=CARTESIAN_POINT('Ctrl Pts',(-19.8964170484326,17.4416849895688,
-18.1829382485014));
#102547=CARTESIAN_POINT('Ctrl Pts',(-19.8964379230461,17.4416987040959,
-18.1829397626504));
#102548=CARTESIAN_POINT('Ctrl Pts',(-19.8964792864155,17.4417258806912,
-18.1829427630446));
#102549=CARTESIAN_POINT('Ctrl Pts',(-19.896499775309,17.4417393428306,-18.1829442492981));
#102550=CARTESIAN_POINT('Ctrl Pts',(-19.8965403902076,17.4417660296852,
-18.1829471955629));
#102551=CARTESIAN_POINT('Ctrl Pts',(-19.8965605160865,17.4417792542996,
-18.1829486555635));
#102552=CARTESIAN_POINT('Ctrl Pts',(-19.8966004260652,17.4418054799222,
-18.1829515508495));
#102553=CARTESIAN_POINT('Ctrl Pts',(-19.8966202100444,17.4418184808345,
-18.1829529861248));
#102554=CARTESIAN_POINT('Ctrl Pts',(-19.8966594552758,17.4418442715238,
-18.1829558333384));
#102555=CARTESIAN_POINT('Ctrl Pts',(-19.8966789167048,17.4418570614016,
-18.1829572452882));
#102556=CARTESIAN_POINT('Ctrl Pts',(-19.8967175357825,17.441882442428,-18.1829600472218));
#102557=CARTESIAN_POINT('Ctrl Pts',(-19.8967366932362,17.4418950334342,
-18.1829614371902));
#102558=CARTESIAN_POINT('Ctrl Pts',(-19.8967747204561,17.441920027252,-18.1829641963253));
#102559=CARTESIAN_POINT('Ctrl Pts',(-19.8967935905899,17.4419324302919,
-18.1829655655174));
#102560=CARTESIAN_POINT('Ctrl Pts',(-19.8968310602207,17.441957059345,-18.1829682843338));
#102561=CARTESIAN_POINT('Ctrl Pts',(-19.8968496593935,17.4419692851327,
-18.1829696339336));
#102562=CARTESIAN_POINT('Ctrl Pts',(-19.8968866015324,17.4419935691303,
-18.1829723146094));
#102563=CARTESIAN_POINT('Ctrl Pts',(-19.8969049445855,17.4420056273859,
-18.1829736456908));
#102564=CARTESIAN_POINT('Ctrl Pts',(-19.8969413887515,17.4420295856634,
-18.1829762903623));
#102565=CARTESIAN_POINT('Ctrl Pts',(-19.8969594898772,17.4420414856832,
-18.1829776039525));
#102566=CARTESIAN_POINT('Ctrl Pts',(-19.8969954631084,17.4420651359514,
-18.1829802145768));
#102567=CARTESIAN_POINT('Ctrl Pts',(-19.897013335426,17.4420768863292,-18.1829815116254));
#102568=CARTESIAN_POINT('Ctrl Pts',(-19.8970488639132,17.4421002457469,
-18.1829840900982));
#102569=CARTESIAN_POINT('Ctrl Pts',(-19.8970665200289,17.4421118547419,
-18.1829853715177));
#102570=CARTESIAN_POINT('Ctrl Pts',(-19.8971016279526,17.4421349391516,
-18.1829879195895));
#102571=CARTESIAN_POINT('Ctrl Pts',(-19.897119079708,17.4421464145228,-18.1829891862372));
#102572=CARTESIAN_POINT('Ctrl Pts',(-19.8971537899676,17.4421692389291,
-18.1829917055657));
#102573=CARTESIAN_POINT('Ctrl Pts',(-19.8971710484817,17.4421805879625,
-18.1829929582466));
#102574=CARTESIAN_POINT('Ctrl Pts',(-19.8972053830992,17.4422031667976,
-18.1829954504262));
#102575=CARTESIAN_POINT('Ctrl Pts',(-19.8972224590889,17.442214396517,-18.1829966899162));
#102576=CARTESIAN_POINT('Ctrl Pts',(-19.8972564383126,17.4422367430508,
-18.1829991564131));
#102577=CARTESIAN_POINT('Ctrl Pts',(-19.8972733416852,17.4422478599493,
-18.1830003834295));
#102578=CARTESIAN_POINT('Ctrl Pts',(-19.8973069854023,17.442269987218,-18.1830028256838));
#102579=CARTESIAN_POINT('Ctrl Pts',(-19.8973237257178,17.4422809975625,
-18.183004040919));
#102580=CARTESIAN_POINT('Ctrl Pts',(-19.8973570527172,17.4423029178835,
-18.1830064602913));
#102581=CARTESIAN_POINT('Ctrl Pts',(-19.8973736392493,17.442313827754,-18.1830076644169));
#102582=CARTESIAN_POINT('Ctrl Pts',(-19.8974066666262,17.4423355523342,
-18.1830100621453));
#102583=CARTESIAN_POINT('Ctrl Pts',(-19.897423107775,17.4423463672379,-18.1830112557697));
#102584=CARTESIAN_POINT('Ctrl Pts',(-19.8974558529991,17.4423679075333,
-18.1830136331196));
#102585=CARTESIAN_POINT('Ctrl Pts',(-19.8974721570837,17.4423786329256,
-18.1830148168454));
#102586=CARTESIAN_POINT('Ctrl Pts',(-19.8975046361975,17.4423999994567,
-18.1830171749789));
#102587=CARTESIAN_POINT('Ctrl Pts',(-19.8975208111424,17.4424106405348,
-18.1830183493801));
#102588=CARTESIAN_POINT('Ctrl Pts',(-19.9010488516823,17.4447317165572,
-18.1832745125599));
#102589=CARTESIAN_POINT('Ctrl Pts',(-19.9045537927668,17.447052583312,-18.183530204642));
#102590=CARTESIAN_POINT('Ctrl Pts',(-19.9146662813489,17.453792181521,-18.1842713686692));
#102591=CARTESIAN_POINT('Ctrl Pts',(-19.9212557994442,17.4582376523508,
-18.1847585891006));
#102592=CARTESIAN_POINT('Ctrl Pts',(-19.9651742349692,17.4882275328669,
-18.1880336327274));
#102593=CARTESIAN_POINT('Ctrl Pts',(-20.0016984188908,17.5149236401384,
-18.1908920390145));
#102594=CARTESIAN_POINT('Ctrl Pts',(-20.1326696719915,17.6172472167952,
-18.201566640356));
#102595=CARTESIAN_POINT('Ctrl Pts',(-20.2214394250199,17.6997597580939,
-18.2096352593239));
#102596=CARTESIAN_POINT('Ctrl Pts',(-20.3997272059662,17.8964923539837,
-18.2271158178451));
#102597=CARTESIAN_POINT('Ctrl Pts',(-20.4855739095568,18.0132601995372,
-18.2364224381902));
#102598=CARTESIAN_POINT('Ctrl Pts',(-20.566111389986,18.1502165884514,-18.246123913703));
#102599=CARTESIAN_POINT('Ctrl Pts',(-20.573236888791,18.1626196900897,-18.2469927641882));
#102600=CARTESIAN_POINT('Ctrl Pts',(-20.5843753119834,18.1824710732244,
-18.2483681911947));
#102601=CARTESIAN_POINT('Ctrl Pts',(-20.5884701466914,18.1898726687203,
-18.2488777032028));
#102602=CARTESIAN_POINT('Ctrl Pts',(-20.5956126063765,18.2029676583951,
-18.249773373814));
#102603=CARTESIAN_POINT('Ctrl Pts',(-20.5986787282876,18.2086507895718,
-18.2501601898928));
#102604=CARTESIAN_POINT('Ctrl Pts',(-20.6049655425978,18.2204322342301,
-18.2509582030556));
#102605=CARTESIAN_POINT('Ctrl Pts',(-20.6081825385662,18.2265324413498,
-18.2513692654643));
#102606=CARTESIAN_POINT('Ctrl Pts',(-20.6163612988826,18.2422267535564,
-18.2524214299886));
#102607=CARTESIAN_POINT('Ctrl Pts',(-20.6212795907519,18.251843383262,-18.2530609939365));
#102608=CARTESIAN_POINT('Ctrl Pts',(-20.6414807697391,18.2920993416723,
-18.2557173388225));
#102609=CARTESIAN_POINT('Ctrl Pts',(-20.6560933274745,18.3230705305152,
-18.2577106884445));
#102610=CARTESIAN_POINT('Ctrl Pts',(-20.6889342113013,18.3972907919699,
-18.262380301961));
#102611=CARTESIAN_POINT('Ctrl Pts',(-20.706487756653,18.4408166001664,-18.2650344917798));
#102612=CARTESIAN_POINT('Ctrl Pts',(-20.7225806130935,18.4848897155193,
-18.2676549617288));
#102613=CARTESIAN_POINT('Ctrl Pts',(-20.7225806765445,18.484889889291,-18.0457834329553));
#102614=CARTESIAN_POINT('Ctrl Pts',(-20.6985951200092,18.4192012099311,
-18.0412345298138));
#102615=CARTESIAN_POINT('Ctrl Pts',(-20.6713591064839,18.3547130434287,
-18.036607855267));
#102616=CARTESIAN_POINT('Ctrl Pts',(-20.6100060409437,18.227448935695,-18.0272719316093));
#102617=CARTESIAN_POINT('Ctrl Pts',(-20.5758218726607,18.1648334862876,
-18.0225709514097));
#102618=CARTESIAN_POINT('Ctrl Pts',(-20.4890913966248,18.0234447836004,
-18.011794881422));
#102619=CARTESIAN_POINT('Ctrl Pts',(-20.4342892301375,17.9462257578456,
-18.005787549224));
#102620=CARTESIAN_POINT('Ctrl Pts',(-20.361084885175,17.8564764069634,-17.9986728828564));
#102621=CARTESIAN_POINT('Ctrl Pts',(-20.3474241242239,17.8402330487983,
-17.9973791311543));
#102622=CARTESIAN_POINT('Ctrl Pts',(-20.328911847463,17.8188812174145,-17.9956697355559));
#102623=CARTESIAN_POINT('Ctrl Pts',(-20.324276160027,17.8135880196861,-17.9952452354522));
#102624=CARTESIAN_POINT('Ctrl Pts',(-20.3150435150256,17.8031512905271,
-17.9944067364924));
#102625=CARTESIAN_POINT('Ctrl Pts',(-20.3104476374453,17.7980069238265,
-17.9939927000969));
#102626=CARTESIAN_POINT('Ctrl Pts',(-20.301501530191,17.7880911338653,-17.993193177619));
#102627=CARTESIAN_POINT('Ctrl Pts',(-20.2971544606214,17.7833169742058,
-17.9928075651126));
#102628=CARTESIAN_POINT('Ctrl Pts',(-20.2870651929699,17.7723377813853,
-17.9919191768738));
#102629=CARTESIAN_POINT('Ctrl Pts',(-20.2813075066278,17.7661470815407,
-17.9914170670517));
#102630=CARTESIAN_POINT('Ctrl Pts',(-20.2657196142296,17.7495869254381,
-17.9900705803206));
#102631=CARTESIAN_POINT('Ctrl Pts',(-20.2558211518402,17.7392821099702,
-17.9892291439662));
#102632=CARTESIAN_POINT('Ctrl Pts',(-20.1641189056051,17.6457298162365,
-17.9815546374228));
#102633=CARTESIAN_POINT('Ctrl Pts',(-20.0756615354366,17.5692751728815,
-17.9750375279399));
#102634=CARTESIAN_POINT('Ctrl Pts',(-19.8501150346933,17.404801296368,-17.959755147767));
#102635=CARTESIAN_POINT('Ctrl Pts',(-19.7083291484311,17.3245383569685,
-17.9511720259872));
#102636=CARTESIAN_POINT('Ctrl Pts',(-19.5285298595371,17.2484785602851,
-17.9399673976099));
#102637=CARTESIAN_POINT('Ctrl Pts',(-19.4979839399778,17.2363870329634,
-17.9380520963707));
#102638=CARTESIAN_POINT('Ctrl Pts',(-19.4603865151649,17.2225071199732,
-17.9356661433535));
#102639=CARTESIAN_POINT('Ctrl Pts',(-19.4535892950707,17.2200372815341,
-17.9352336646788));
#102640=CARTESIAN_POINT('Ctrl Pts',(-19.4428808250131,17.2162082513649,
-17.9345503685363));
#102641=CARTESIAN_POINT('Ctrl Pts',(-19.4389779416827,17.2148255974089,
-17.9343009216384));
#102642=CARTESIAN_POINT('Ctrl Pts',(-19.4317044484996,17.2122728468447,
-17.933835244512));
#102643=CARTESIAN_POINT('Ctrl Pts',(-19.4283349281391,17.2110998182016,
-17.9336191910398));
#102644=CARTESIAN_POINT('Ctrl Pts',(-19.4206744250733,17.2084546662967,
-17.9331272720577));
#102645=CARTESIAN_POINT('Ctrl Pts',(-19.4163816851902,17.206987820791,-17.9328511001117));
#102646=CARTESIAN_POINT('Ctrl Pts',(-19.403587754782,17.2026619599005,-17.9320265497939));
#102647=CARTESIAN_POINT('Ctrl Pts',(-19.395073199251,17.1998432026886,-17.9314758878544));
#102648=CARTESIAN_POINT('Ctrl Pts',(-19.3293524721863,17.1785486865685,
-17.9272122412649));
#102649=CARTESIAN_POINT('Ctrl Pts',(-19.2714057866816,17.1624647890181,
-17.9233761802053));
#102650=CARTESIAN_POINT('Ctrl Pts',(-19.0646095532864,17.1144434065282,
-17.9095986480423));
#102651=CARTESIAN_POINT('Ctrl Pts',(-18.9130774368891,17.0961033169612,
-17.8993834197686));
#102652=CARTESIAN_POINT('Ctrl Pts',(-18.6951686767517,17.0933362306514,
-17.8852648883115));
#102653=CARTESIAN_POINT('Ctrl Pts',(-18.6294493227224,17.0955619352564,
-17.8810743215709));
#102654=CARTESIAN_POINT('Ctrl Pts',(-18.5382841715414,17.1029092676702,
-17.8753676862236));
#102655=CARTESIAN_POINT('Ctrl Pts',(-18.5126726798799,17.1054441282285,
-17.8737760310758));
#102656=CARTESIAN_POINT('Ctrl Pts',(-18.4682385804139,17.1106616895351,
-17.8710341334243));
#102657=CARTESIAN_POINT('Ctrl Pts',(-18.449394529272,17.1131320552646,-17.8698774440636));
#102658=CARTESIAN_POINT('Ctrl Pts',(-18.4219756719704,17.1171027943525,
-17.8682029035969));
#102659=CARTESIAN_POINT('Ctrl Pts',(-18.4133732116025,17.118402772822,-17.8676787497316));
#102660=CARTESIAN_POINT('Ctrl Pts',(-18.3983851880166,17.1207623123725,
-17.8667675802522));
#102661=CARTESIAN_POINT('Ctrl Pts',(-18.3919960637012,17.1217981902648,
-17.8663798197476));
#102662=CARTESIAN_POINT('Ctrl Pts',(-18.3796570304333,17.123856855543,-17.8656321849995));
#102663=CARTESIAN_POINT('Ctrl Pts',(-18.3737065559855,17.1248758232317,
-17.8652721936421));
#102664=CARTESIAN_POINT('Ctrl Pts',(-18.3595833261947,17.1273565364797,
-17.8644190447225));
#102665=CARTESIAN_POINT('Ctrl Pts',(-18.3514146116188,17.1288409397269,
-17.8639266110314));
#102666=CARTESIAN_POINT('Ctrl Pts',(-18.3224743261575,17.1342759749742,
-17.8621854505945));
#102667=CARTESIAN_POINT('Ctrl Pts',(-18.3017530076761,17.1384897728596,
-17.8609450944425));
#102668=CARTESIAN_POINT('Ctrl Pts',(-18.0916287167026,17.1845083349567,
-17.8484221103672));
#102669=CARTESIAN_POINT('Ctrl Pts',(-17.9087686838356,17.2518400501761,
-17.838091247687));
#102670=CARTESIAN_POINT('Ctrl Pts',(-17.6716117867266,17.378346812602,-17.8234097502943));
#102671=CARTESIAN_POINT('Ctrl Pts',(-17.6075183318053,17.41703128546,-17.8192802040188));
#102672=CARTESIAN_POINT('Ctrl Pts',(-17.5170123390496,17.4784226366979,
-17.8130147588829));
#102673=CARTESIAN_POINT('Ctrl Pts',(-17.4888937658892,17.4985183381089,
-17.8110023534249));
#102674=CARTESIAN_POINT('Ctrl Pts',(-17.455388180843,17.5237255100739,-17.8085066242993));
#102675=CARTESIAN_POINT('Ctrl Pts',(-17.4495181962696,17.5281898857285,
-17.8080656481993));
#102676=CARTESIAN_POINT('Ctrl Pts',(-17.4403901534224,17.5352077398579,
-17.8073738457691));
#102677=CARTESIAN_POINT('Ctrl Pts',(-17.4371159894631,17.5377403080053,
-17.8071244716997));
#102678=CARTESIAN_POINT('Ctrl Pts',(-17.4310334042903,17.5424737695482,
-17.8066588582191));
#102679=CARTESIAN_POINT('Ctrl Pts',(-17.4282231122649,17.5446721660874,
-17.8064427951141));
#102680=CARTESIAN_POINT('Ctrl Pts',(-17.4218510184215,17.5496828582446,
-17.8059507598805));
#102681=CARTESIAN_POINT('Ctrl Pts',(-17.4182927095791,17.5524994964141,
-17.8056744807194));
#102682=CARTESIAN_POINT('Ctrl Pts',(-17.4077225426793,17.5609219116814,
-17.8048493201447));
#102683=CARTESIAN_POINT('Ctrl Pts',(-17.4007373596164,17.5665607896425,
-17.8042981502665));
#102684=CARTESIAN_POINT('Ctrl Pts',(-17.3470609360387,17.6104585739092,
-17.800018609476));
#102685=CARTESIAN_POINT('Ctrl Pts',(-17.3019937264599,17.6506508648063,
-17.7961661517238));
#102686=CARTESIAN_POINT('Ctrl Pts',(-17.1528658178934,17.7955552030458,
-17.7826699821423));
#102687=CARTESIAN_POINT('Ctrl Pts',(-17.0580649604111,17.9091879598663,
-17.7727712742713));
#102688=CARTESIAN_POINT('Ctrl Pts',(-16.9186473011171,18.1170487009912,
-17.7565251032165));
#102689=CARTESIAN_POINT('Ctrl Pts',(-16.8677190120586,18.206392833318,-17.7500258788693));
#102690=CARTESIAN_POINT('Ctrl Pts',(-16.8170973498081,18.3124499183923,
-17.7428593430256));
#102691=CARTESIAN_POINT('Ctrl Pts',(-16.8108625941288,18.325872576935,-17.7419617195481));
#102692=CARTESIAN_POINT('Ctrl Pts',(-16.8015710638977,18.3464378377419,
-17.740600425083));
#102693=CARTESIAN_POINT('Ctrl Pts',(-16.7984120934352,18.3535335085488,
-17.7401332474842));
#102694=CARTESIAN_POINT('Ctrl Pts',(-16.7927370135165,18.3664720351234,
-17.7392858826598));
#102695=CARTESIAN_POINT('Ctrl Pts',(-16.7902080645199,18.3723091278191,
-17.7389052593423));
#102696=CARTESIAN_POINT('Ctrl Pts',(-16.7848064214292,18.3849323904007,
-17.7380856562206));
#102697=CARTESIAN_POINT('Ctrl Pts',(-16.7819427658821,18.3917223552396,
-17.7376469882315));
#102698=CARTESIAN_POINT('Ctrl Pts',(-16.7742770997471,18.4101666636094,
-17.7364612273543));
#102699=CARTESIAN_POINT('Ctrl Pts',(-16.7695435781595,18.4218492821528,
-17.7357164582436));
#102700=CARTESIAN_POINT('Ctrl Pts',(-16.747061600226,18.4787922142323,-17.7321159094484));
#102701=CARTESIAN_POINT('Ctrl Pts',(-16.7307706102398,18.5246145458371,
-17.7293092478705));
#102702=CARTESIAN_POINT('Ctrl Pts',(-16.7037373127509,18.6098455860685,
-17.7242274497607));
#102703=CARTESIAN_POINT('Ctrl Pts',(-16.6925298605576,18.6490808565139,
-17.7219404679047));
#102704=CARTESIAN_POINT('Ctrl Pts',(-16.64929393253,18.8188798706058,-17.7122163846758));
#102705=CARTESIAN_POINT('Ctrl Pts',(-16.6286077305665,18.9520014028685,
-17.7050482410997));
#102706=CARTESIAN_POINT('Ctrl Pts',(-16.6169859545199,19.148775679534,-17.6942149502253));
#102707=CARTESIAN_POINT('Ctrl Pts',(-16.6160720171754,19.2114959085012,
-17.6907228035505));
#102708=CARTESIAN_POINT('Ctrl Pts',(-16.6188649731704,19.3050698584071,
-17.6853380267219));
#102709=CARTESIAN_POINT('Ctrl Pts',(-16.6204647157198,19.3359547721859,
-17.6835321195927));
#102710=CARTESIAN_POINT('Ctrl Pts',(-16.6232647715201,19.3739006052262,
-17.6812660780505));
#102711=CARTESIAN_POINT('Ctrl Pts',(-16.6238252382374,19.3810067159219,
-17.6808396716993));
#102712=CARTESIAN_POINT('Ctrl Pts',(-16.6247633415222,19.3921805926096,
-17.6801657690125));
#102713=CARTESIAN_POINT('Ctrl Pts',(-16.6251168889131,19.3962504027756,
-17.6799196046971));
#102714=CARTESIAN_POINT('Ctrl Pts',(-16.6258019820485,19.4038805408688,
-17.6794567146712));
#102715=CARTESIAN_POINT('Ctrl Pts',(-16.6261307690229,19.4074410607812,
-17.6792401451599));
#102716=CARTESIAN_POINT('Ctrl Pts',(-16.626904994002,19.4155995489266,-17.6787426138371));
#102717=CARTESIAN_POINT('Ctrl Pts',(-16.6273564611378,19.4201968904136,
-17.6784613171599));
#102718=CARTESIAN_POINT('Ctrl Pts',(-16.6288020339352,19.4344379411968,
-17.677587129888));
#102719=CARTESIAN_POINT('Ctrl Pts',(-16.6298473244732,19.4440761672906,
-17.6769914736153));
#102720=CARTESIAN_POINT('Ctrl Pts',(-16.6423861071656,19.552724100822,-17.6702341536958));
#102721=CARTESIAN_POINT('Ctrl Pts',(-16.6607910025215,19.650799697077,-17.6637390136366));
#102722=CARTESIAN_POINT('Ctrl Pts',(-16.715531310881,19.8598750215869,-17.6495000049824));
#102723=CARTESIAN_POINT('Ctrl Pts',(-16.7542821631584,19.9699302654033,
-17.641760308951));
#102724=CARTESIAN_POINT('Ctrl Pts',(-16.8274376647242,20.1332884303513,
-17.6301901867847));
#102725=CARTESIAN_POINT('Ctrl Pts',(-16.8554998142507,20.1891789740647,
-17.626212585505));
#102726=CARTESIAN_POINT('Ctrl Pts',(-16.904317991302,20.2765342442579,-17.6199755853184));
#102727=CARTESIAN_POINT('Ctrl Pts',(-16.9235093489325,20.3088266549785,
-17.6176649915191));
#102728=CARTESIAN_POINT('Ctrl Pts',(-16.9495089489827,20.3500370396981,
-17.6147077975544));
#102729=CARTESIAN_POINT('Ctrl Pts',(-16.9555418644964,20.3594338712831,
-17.6140328915913));
#102730=CARTESIAN_POINT('Ctrl Pts',(-16.9654645930722,20.3746237328452,
-17.6129408024179));
#102731=CARTESIAN_POINT('Ctrl Pts',(-16.9693091337935,20.3804459481904,
-17.6125219399504));
#102732=CARTESIAN_POINT('Ctrl Pts',(-16.9767512074393,20.3915960388531,
-17.6117192175117));
#102733=CARTESIAN_POINT('Ctrl Pts',(-16.9803443580061,20.3969267332437,
-17.6113351988377));
#102734=CARTESIAN_POINT('Ctrl Pts',(-16.9886176291906,20.409080899034,-17.6104590075412));
#102735=CARTESIAN_POINT('Ctrl Pts',(-16.9933136022126,20.4158934925906,
-17.6099674420141));
#102736=CARTESIAN_POINT('Ctrl Pts',(-17.0058745942221,20.4338894063995,
-17.6086676261772));
#102737=CARTESIAN_POINT('Ctrl Pts',(-17.0138082928204,20.4450244819346,
-17.6078620024366));
#102738=CARTESIAN_POINT('Ctrl Pts',(-17.0737687035965,20.5274778792088,
-17.6018845299312));
#102739=CARTESIAN_POINT('Ctrl Pts',(-17.1301061482496,20.5955610073797,
-17.5968867281685));
#102740=CARTESIAN_POINT('Ctrl Pts',(-17.2865870583059,20.7622508795801,
-17.5842174296299));
#102741=CARTESIAN_POINT('Ctrl Pts',(-17.3925690089595,20.8547593171523,
-17.576753249044));
#102742=CARTESIAN_POINT('Ctrl Pts',(-17.5527036666521,20.9686644804882,
-17.5659056486565));
#102743=CARTESIAN_POINT('Ctrl Pts',(-17.5997605933034,20.9993918859522,
-17.5627599921487));
#102744=CARTESIAN_POINT('Ctrl Pts',(-17.6726904283673,21.0429769854792,
-17.5578610120988));
#102745=CARTESIAN_POINT('Ctrl Pts',(-17.69769800557,21.0572382492745,-17.5561770558546));
#102746=CARTESIAN_POINT('Ctrl Pts',(-17.7291086790429,21.0743118306277,
-17.5540470883347));
#102747=CARTESIAN_POINT('Ctrl Pts',(-17.7352465173272,21.0776089635654,
-17.5536301869386));
#102748=CARTESIAN_POINT('Ctrl Pts',(-17.744977300651,21.0827744253641,-17.552967971154));
#102749=CARTESIAN_POINT('Ctrl Pts',(-17.7485595854915,21.0846628800549,
-17.5527239127521));
#102750=CARTESIAN_POINT('Ctrl Pts',(-17.7553209733597,21.0882024919853,
-17.5522627134764));
#102751=CARTESIAN_POINT('Ctrl Pts',(-17.7584988567404,21.0898558624569,
-17.5520457152807));
#102752=CARTESIAN_POINT('Ctrl Pts',(-17.7657675796006,21.0936141787162,
-17.5515488612772));
#102753=CARTESIAN_POINT('Ctrl Pts',(-17.7698610888007,21.0957138575405,
-17.5512686790194));
#102754=CARTESIAN_POINT('Ctrl Pts',(-17.7807336208873,21.1012460019208,
-17.5505235888855));
#102755=CARTESIAN_POINT('Ctrl Pts',(-17.7875242640531,21.1046553051206,
-17.5500572899114));
#102756=CARTESIAN_POINT('Ctrl Pts',(-17.8348275142629,21.1280863273992,
-17.54680333902));
#102757=CARTESIAN_POINT('Ctrl Pts',(-17.8759507443142,21.1468414080146,
-17.5439455470446));
#102758=CARTESIAN_POINT('Ctrl Pts',(-17.9231850083496,21.1665828239092,
-17.5406558110589));
#102759=CARTESIAN_POINT('Ctrl Pts',(-17.9287408809804,21.1688771365707,
-17.5402687445102));
#102760=CARTESIAN_POINT('Ctrl Pts',(-18.080145808931,21.2306467415208,-17.5297188583977));
#102761=CARTESIAN_POINT('Ctrl Pts',(-18.2321701161883,21.2736848361996,
-17.5191274540402));
#102762=CARTESIAN_POINT('Ctrl Pts',(-18.4891774617685,21.3163169586241,
-17.502214753407));
#102763=CARTESIAN_POINT('Ctrl Pts',(-18.5918926189619,21.3257360424972,
-17.4956954335792));
#102764=CARTESIAN_POINT('Ctrl Pts',(-18.7097044899123,21.327912372036,-17.4885097256611));
#102765=CARTESIAN_POINT('Ctrl Pts',(-18.7245122324675,21.3280305294063,
-17.4876115975902));
#102766=CARTESIAN_POINT('Ctrl Pts',(-18.747088938308,21.327973791018,-17.4862496984533));
#102767=CARTESIAN_POINT('Ctrl Pts',(-18.7548574922321,21.3279115049266,
-17.4857824159939));
#102768=CARTESIAN_POINT('Ctrl Pts',(-18.7689864179481,21.3277204392288,
-17.4849349404553));
#102769=CARTESIAN_POINT('Ctrl Pts',(-18.7753468598717,21.3276057511583,
-17.4845543107185));
#102770=CARTESIAN_POINT('Ctrl Pts',(-18.7890725087859,21.3272963641361,
-17.483734782192));
#102771=CARTESIAN_POINT('Ctrl Pts',(-18.796437428351,21.327091881683,-17.4832961947411));
#102772=CARTESIAN_POINT('Ctrl Pts',(-18.8163930810902,21.3264335508718,
-17.4821108656093));
#102773=CARTESIAN_POINT('Ctrl Pts',(-18.8289811992942,21.3259057449613,
-17.4813664448226));
#102774=CARTESIAN_POINT('Ctrl Pts',(-18.8900493571073,21.3227988792562,
-17.4777701752275));
#102775=CARTESIAN_POINT('Ctrl Pts',(-18.9384378558316,21.3186649645855,
-17.4749673007283));
#102776=CARTESIAN_POINT('Ctrl Pts',(-19.0271581928347,21.3080008014141,
-17.4698884559444));
#102777=CARTESIAN_POINT('Ctrl Pts',(-19.067524120617,21.3019605433582,-17.4676007725183));
#102778=CARTESIAN_POINT('Ctrl Pts',(-19.2400316756001,21.2710237990694,
-17.4578740025092));
#102779=CARTESIAN_POINT('Ctrl Pts',(-19.3698054401631,21.2347383362235,
-17.4507041686132));
#102780=CARTESIAN_POINT('Ctrl Pts',(-19.5537914738126,21.1638352688755,
-17.4398678578979));
#102781=CARTESIAN_POINT('Ctrl Pts',(-19.6112868413681,21.1386904046713,
-17.4363743124226));
#102782=CARTESIAN_POINT('Ctrl Pts',(-19.6953392007928,21.0973914704745,
-17.4309875850741));
#102783=CARTESIAN_POINT('Ctrl Pts',(-19.7227978203557,21.0831443539837,
-17.4291812000981));
#102784=CARTESIAN_POINT('Ctrl Pts',(-19.7561871347506,21.0648806008284,
-17.4269146260797));
#102785=CARTESIAN_POINT('Ctrl Pts',(-19.7624240518356,21.0614280010019,
-17.4264881838816));
#102786=CARTESIAN_POINT('Ctrl Pts',(-19.7722074697831,21.055947408298,-17.4258142371316));
#102787=CARTESIAN_POINT('Ctrl Pts',(-19.7757658076228,21.0539405012419,
-17.4255680648901));
#102788=CARTESIAN_POINT('Ctrl Pts',(-19.7824276929388,21.050157730718,-17.4251051683479));
#102789=CARTESIAN_POINT('Ctrl Pts',(-19.785532557818,21.0483842997452,-17.4248886002967));
#102790=CARTESIAN_POINT('Ctrl Pts',(-19.7926381769983,21.0443018158387,
-17.4243910835013));
#102791=CARTESIAN_POINT('Ctrl Pts',(-19.7966358651826,21.0419875354163,
-17.4241097999639));
#102792=CARTESIAN_POINT('Ctrl Pts',(-19.808999337092,21.0347761359002,-17.42323569332));
#102793=CARTESIAN_POINT('Ctrl Pts',(-19.8173389445984,21.0298347070425,
-17.4226401052558));
#102794=CARTESIAN_POINT('Ctrl Pts',(-19.9078136176254,20.9753831851072,
-17.4161158807588));
#102795=CARTESIAN_POINT('Ctrl Pts',(-19.9865184503359,20.9204091419468,
-17.4098781014981));
#102796=CARTESIAN_POINT('Ctrl Pts',(-20.1599363469923,20.7808570304567,
-17.3952250866863));
#102797=CARTESIAN_POINT('Ctrl Pts',(-20.2513329036141,20.6927053916774,
-17.3867950043775));
#102798=CARTESIAN_POINT('Ctrl Pts',(-20.3724509589717,20.552850896293,-17.3748732027538));
#102799=CARTESIAN_POINT('Ctrl Pts',(-20.4087702461443,20.5072372297808,
-17.3711748545664));
#102800=CARTESIAN_POINT('Ctrl Pts',(-20.4642424642891,20.43133853269,-17.3653244785605));
#102801=CARTESIAN_POINT('Ctrl Pts',(-20.4845890000875,20.4019674707893,
-17.3631287712228));
#102802=CARTESIAN_POINT('Ctrl Pts',(-20.5101992674296,20.362922510238,-17.3602957191564));
#102803=CARTESIAN_POINT('Ctrl Pts',(-20.5161437703807,20.3537042031934,
-17.3596329248477));
#102804=CARTESIAN_POINT('Ctrl Pts',(-20.5257284845305,20.3385841907032,
-17.3585555425984));
#102805=CARTESIAN_POINT('Ctrl Pts',(-20.5294117639498,20.3327101537616,
-17.3581393588845));
#102806=CARTESIAN_POINT('Ctrl Pts',(-20.5364622496124,20.3213424492668,
-17.3573384630007));
#102807=CARTESIAN_POINT('Ctrl Pts',(-20.5398333574654,20.3158513033001,
-17.3569536098317));
#102808=CARTESIAN_POINT('Ctrl Pts',(-20.5475262959706,20.3031911209873,
-17.3560708879837));
#102809=CARTESIAN_POINT('Ctrl Pts',(-20.5518307988009,20.2960116409249,
-17.3555736579241));
#102810=CARTESIAN_POINT('Ctrl Pts',(-20.5632212069067,20.2767555181233,
-17.3542488382614));
#102811=CARTESIAN_POINT('Ctrl Pts',(-20.5702301503391,20.2646336636768,
-17.3534240412733));
#102812=CARTESIAN_POINT('Ctrl Pts',(-20.6269890232292,20.1641832970636,
-17.3466623069611));
#102813=CARTESIAN_POINT('Ctrl Pts',(-20.6704590839962,20.0724498634047,
-17.3409589440621));
#102814=CARTESIAN_POINT('Ctrl Pts',(-20.7617045426689,19.8376937515129,
-17.3270883305746));
#102815=CARTESIAN_POINT('Ctrl Pts',(-20.801105109675,19.6920424586304,-17.3191197810486));
#102816=CARTESIAN_POINT('Ctrl Pts',(-20.8309456068991,19.504382681921,-17.3084711625934));
#102817=CARTESIAN_POINT('Ctrl Pts',(-20.8360618079081,19.4651457553009,
-17.3062221924579));
#102818=CARTESIAN_POINT('Ctrl Pts',(-20.8416060196543,19.4107834663772,
-17.3030475437583));
#102819=CARTESIAN_POINT('Ctrl Pts',(-20.8429760799789,19.3957604796477,
-17.3021640596538));
#102820=CARTESIAN_POINT('Ctrl Pts',(-20.8450676744407,19.3697556892886,
-17.3006221200066));
#102821=CARTESIAN_POINT('Ctrl Pts',(-20.8458643545028,19.3587803486912,
-17.2999674604093));
#102822=CARTESIAN_POINT('Ctrl Pts',(-20.8468897379978,19.3429455029684,
-17.2990167057978));
#102823=CARTESIAN_POINT('Ctrl Pts',(-20.8471873277521,19.338090430167,-17.2987243535215));
#102824=CARTESIAN_POINT('Ctrl Pts',(-20.8476764825848,19.3296328035305,
-17.29821353356));
#102825=CARTESIAN_POINT('Ctrl Pts',(-20.8478755777301,19.3260306778402,
-17.2979954875501));
#102826=CARTESIAN_POINT('Ctrl Pts',(-20.8482735902958,19.3184793960689,
-17.2975373444059));
#102827=CARTESIAN_POINT('Ctrl Pts',(-20.8484706505186,19.3145302018941,
-17.2972971491645));
#102828=CARTESIAN_POINT('Ctrl Pts',(-20.8489642021392,19.3040493141564,
-17.2966581533865));
#102829=CARTESIAN_POINT('Ctrl Pts',(-20.8492414964717,19.2975168204044,
-17.2962583014388));
#102830=CARTESIAN_POINT('Ctrl Pts',(-20.8502933314452,19.2696966842009,
-17.29454901154));
#102831=CARTESIAN_POINT('Ctrl Pts',(-20.8507767753518,19.2484001129417,
-17.2932245199956));
#102832=CARTESIAN_POINT('Ctrl Pts',(-20.8509781232099,19.2219268983958,
-17.2915611593869));
#102833=CARTESIAN_POINT('Ctrl Pts',(-20.850998506442,19.216752877949,-17.2912352624917));
#102834=CARTESIAN_POINT('Ctrl Pts',(-20.8510131828748,19.1630721313074,
-17.287846074883));
#102835=CARTESIAN_POINT('Ctrl Pts',(-20.8493592891271,19.1145823847139,
-17.284717231432));
#102836=CARTESIAN_POINT('Ctrl Pts',(-20.8326138661285,18.8703421985657,
-17.2687465213729));
#102837=CARTESIAN_POINT('Ctrl Pts',(-20.7920024891764,18.6772600447215,
-17.2555538816513));
#102838=CARTESIAN_POINT('Ctrl Pts',(-20.7244363838141,18.4899872681561,
-17.2430396061983));
#102839=CARTESIAN_POINT('Ctrl Pts',(-20.723510942024,18.4874375847904,-17.2428692571384));
#102840=CARTESIAN_POINT('Ctrl Pts',(-20.7225806138883,18.484889717696,-17.2426990599955));
#102841=CARTESIAN_POINT('Origin',(-18.734,19.211,0.));
#102842=CARTESIAN_POINT('',(-20.7225806308032,18.4848897640204,-16.4437314734851));
#102843=CARTESIAN_POINT('',(-20.7225806137285,18.4848897172584,-16.6645990097762));
#102844=CARTESIAN_POINT('',(-20.7225806137986,18.4848897174502,0.));
#102845=CARTESIAN_POINT('',(-20.850999201232,19.209903974194,-16.7126929569557));
#102846=CARTESIAN_POINT('Ctrl Pts',(-20.7225806137285,18.4848897172584,
-16.6645990097762));
#102847=CARTESIAN_POINT('Ctrl Pts',(-20.7243922735201,18.4898512659733,
-16.6649340211793));
#102848=CARTESIAN_POINT('Ctrl Pts',(-20.7261853754752,18.4948196247617,
-16.665269794044));
#102849=CARTESIAN_POINT('Ctrl Pts',(-20.7539879299496,18.5727678309291,
-16.6705418857637));
#102850=CARTESIAN_POINT('Ctrl Pts',(-20.7759887406123,18.6471100343595,
-16.6756251051418));
#102851=CARTESIAN_POINT('Ctrl Pts',(-20.8317361364545,18.8821735502559,
-16.6915678158184));
#102852=CARTESIAN_POINT('Ctrl Pts',(-20.8509145479737,19.0457465062896,
-16.7024244527962));
#102853=CARTESIAN_POINT('Ctrl Pts',(-20.8509997150783,19.2099016565369,
-16.7126937055852));
#102854=CARTESIAN_POINT('Ctrl Pts',(-20.8509997162505,19.2099039182537,
-16.7126938470741));
#102855=CARTESIAN_POINT('Ctrl Pts',(-20.8510131380481,19.2358271139468,
-16.714315555052));
#102856=CARTESIAN_POINT('Ctrl Pts',(-20.8505504063664,19.2617494365499,
-16.7159232464005));
#102857=CARTESIAN_POINT('Ctrl Pts',(-20.8489736684266,19.3052644117491,
-16.7185990200433));
#102858=CARTESIAN_POINT('Ctrl Pts',(-20.8481159290052,19.3228627088576,
-16.7196748359838));
#102859=CARTESIAN_POINT('Ctrl Pts',(-20.8465415719745,19.3485615206045,
-16.7212369315558));
#102860=CARTESIAN_POINT('Ctrl Pts',(-20.8459978398512,19.3566715230364,
-16.7217285975398));
#102861=CARTESIAN_POINT('Ctrl Pts',(-20.84495266486,19.3710219903606,-16.7225963419054));
#102862=CARTESIAN_POINT('Ctrl Pts',(-20.8444702256611,19.3772637019614,
-16.7229730125008));
#102863=CARTESIAN_POINT('Ctrl Pts',(-20.8434611332646,19.3896063383327,
-16.7237163971605));
#102864=CARTESIAN_POINT('Ctrl Pts',(-20.8429356823552,19.3957072975211,
-16.7240831452476));
#102865=CARTESIAN_POINT('Ctrl Pts',(-20.8418361329149,19.4078571927139,
-16.724812137682));
#102866=CARTESIAN_POINT('Ctrl Pts',(-20.841262449406,19.4139061064936,-16.7251743913984));
#102867=CARTESIAN_POINT('Ctrl Pts',(-20.8398285581254,19.4283626221666,
-16.7260385677845));
#102868=CARTESIAN_POINT('Ctrl Pts',(-20.838944025948,19.4367677490365,-16.7265397217195));
#102869=CARTESIAN_POINT('Ctrl Pts',(-20.8360988515349,19.4623318192594,
-16.7280602165821));
#102870=CARTESIAN_POINT('Ctrl Pts',(-20.8339785214729,19.4794725319764,
-16.7290745437001));
#102871=CARTESIAN_POINT('Ctrl Pts',(-20.8260338095488,19.5378270308262,
-16.7325118514138));
#102872=CARTESIAN_POINT('Ctrl Pts',(-20.8192037326319,19.5788954855934,
-16.7349035867475));
#102873=CARTESIAN_POINT('Ctrl Pts',(-20.7779734636126,19.7884237590213,
-16.7470133767205));
#102874=CARTESIAN_POINT('Ctrl Pts',(-20.7243586254664,19.9524297643781,
-16.7561209403142));
#102875=CARTESIAN_POINT('Ctrl Pts',(-20.6249328324955,20.1649353425292,
-16.7690150952559));
#102876=CARTESIAN_POINT('Ctrl Pts',(-20.5958562969027,20.220509582028,-16.7725069378238));
#102877=CARTESIAN_POINT('Ctrl Pts',(-20.5488220085098,20.3014431597294,
-16.7778912905825));
#102878=CARTESIAN_POINT('Ctrl Pts',(-20.5327016379616,20.3278336482267,
-16.7796970938042));
#102879=CARTESIAN_POINT('Ctrl Pts',(-20.5121619834855,20.3598602049572,
-16.7819630195547));
#102880=CARTESIAN_POINT('Ctrl Pts',(-20.5082836600394,20.365840811746,-16.7823894181052));
#102881=CARTESIAN_POINT('Ctrl Pts',(-20.5021352904952,20.3752178846214,
-16.7830633112008));
#102882=CARTESIAN_POINT('Ctrl Pts',(-20.4998854488861,20.3786276243436,
-16.7833094737889));
#102883=CARTESIAN_POINT('Ctrl Pts',(-20.4956478283573,20.3850096740737,
-16.7837723623906));
#102884=CARTESIAN_POINT('Ctrl Pts',(-20.4936623833385,20.387983467156,-16.783988932216));
#102885=CARTESIAN_POINT('Ctrl Pts',(-20.4890946289215,20.3947876429835,
-16.7844864666896));
#102886=CARTESIAN_POINT('Ctrl Pts',(-20.486507317039,20.3986146020239,-16.7847677662195));
#102887=CARTESIAN_POINT('Ctrl Pts',(-20.4784512063112,20.410446948935,-16.7856419710095));
#102888=CARTESIAN_POINT('Ctrl Pts',(-20.4729400153029,20.4184231277742,
-16.7862376421043));
#102889=CARTESIAN_POINT('Ctrl Pts',(-20.4106715035772,20.5072318371383,
-16.7929390210152));
#102890=CARTESIAN_POINT('Ctrl Pts',(-20.3483849501997,20.5840261871356,
-16.7993722827136));
#102891=CARTESIAN_POINT('Ctrl Pts',(-20.1664593466636,20.7787658150669,
-16.8169267314158));
#102892=CARTESIAN_POINT('Ctrl Pts',(-20.0377573938488,20.887324133974,-16.8280724350466));
#102893=CARTESIAN_POINT('Ctrl Pts',(-19.8712093579943,20.9969003370978,
-16.8405985891722));
#102894=CARTESIAN_POINT('Ctrl Pts',(-19.8444569268267,21.0136565720525,
-16.8425612093817));
#102895=CARTESIAN_POINT('Ctrl Pts',(-19.8041717197435,21.0376516814561,
-16.845444733301));
#102896=CARTESIAN_POINT('Ctrl Pts',(-19.790919746447,21.0453512597232,-16.8463820414283));
#102897=CARTESIAN_POINT('Ctrl Pts',(-19.7666473240213,21.0591034986998,
-16.8480787412602));
#102898=CARTESIAN_POINT('Ctrl Pts',(-19.7556544347017,21.0652031346264,
-16.8488397949379));
#102899=CARTESIAN_POINT('Ctrl Pts',(-19.738262448279,21.0746518130283,-16.8500324793849));
#102900=CARTESIAN_POINT('Ctrl Pts',(-19.7318995651862,21.0780665775593,
-16.8504664503689));
#102901=CARTESIAN_POINT('Ctrl Pts',(-19.7254731420198,21.0814732052019,
-16.8509023944279));
#102902=CARTESIAN_POINT('Ctrl Pts',(-19.7254270100311,21.0814976574446,
-16.850905523724));
#102903=CARTESIAN_POINT('Ctrl Pts',(-19.7253331200524,21.0815474193421,
-16.8509118923652));
#102904=CARTESIAN_POINT('Ctrl Pts',(-19.7252853607656,21.0815727295276,
-16.8509151317894));
#102905=CARTESIAN_POINT('Ctrl Pts',(-19.7251881569115,21.08162423825,-16.8509217246807));
#102906=CARTESIAN_POINT('Ctrl Pts',(-19.7251387113115,21.0816504371662,
-16.8509250782086));
#102907=CARTESIAN_POINT('Ctrl Pts',(-19.7250380730387,21.0817037555805,
-16.8509319034698));
#102908=CARTESIAN_POINT('Ctrl Pts',(-19.7249868797228,21.081730875239,-16.8509353752367));
#102909=CARTESIAN_POINT('Ctrl Pts',(-19.7248826823109,21.0817860683394,
-16.8509424412658));
#102910=CARTESIAN_POINT('Ctrl Pts',(-19.7248296773664,21.0818141420373,
-16.8509460355747));
#102911=CARTESIAN_POINT('Ctrl Pts',(-19.724721790746,21.0818712775594,-16.8509533511273));
#102912=CARTESIAN_POINT('Ctrl Pts',(-19.7246669081625,21.0819003396568,
-16.8509570724209));
#102913=CARTESIAN_POINT('Ctrl Pts',(-19.7245551977369,21.0819594876347,
-16.8509646465542));
#102914=CARTESIAN_POINT('Ctrl Pts',(-19.7244983690897,21.0819895737188,
-16.850968499436));
#102915=CARTESIAN_POINT('Ctrl Pts',(-19.7243826953439,21.0820508066848,
-16.8509763415345));
#102916=CARTESIAN_POINT('Ctrl Pts',(-19.7243238497194,21.0820819536058,
-16.8509803307736));
#102917=CARTESIAN_POINT('Ctrl Pts',(-19.7242040684595,21.0821453464546,
-16.8509884505331));
#102918=CARTESIAN_POINT('Ctrl Pts',(-19.7241431321865,21.0821775924632,
-16.8509925810823));
#102919=CARTESIAN_POINT('Ctrl Pts',(-19.7240190935729,21.0822432229556,
-16.851000988574));
#102920=CARTESIAN_POINT('Ctrl Pts',(-19.7239559904609,21.0822766075722,
-16.8510052655535));
#102921=CARTESIAN_POINT('Ctrl Pts',(-19.7238275390494,21.0823445563028,
-16.8510139712215));
#102922=CARTESIAN_POINT('Ctrl Pts',(-19.7237621903787,21.0823791203179,
-16.8510183999188));
#102923=CARTESIAN_POINT('Ctrl Pts',(-19.7236291640709,21.0824494712604,
-16.8510274146503));
#102924=CARTESIAN_POINT('Ctrl Pts',(-19.7235614890042,21.0824852565114,
-16.8510320004925));
#102925=CARTESIAN_POINT('Ctrl Pts',(-19.7234348799324,21.0825521961239,
-16.851040579369));
#102926=CARTESIAN_POINT('Ctrl Pts',(-19.7233759451185,21.0825833520483,
-16.8510445725215));
#102927=CARTESIAN_POINT('Ctrl Pts',(-19.7232483244762,21.0826508110639,
-16.8510532190799));
#102928=CARTESIAN_POINT('Ctrl Pts',(-19.7231796369936,21.0826871137539,
-16.8510578725267));
#102929=CARTESIAN_POINT('Ctrl Pts',(-19.7230309145422,21.0827657060309,
-16.8510679476066));
#102930=CARTESIAN_POINT('Ctrl Pts',(-19.7229508780295,21.0828079947042,
-16.8510733692477));
#102931=CARTESIAN_POINT('Ctrl Pts',(-19.722777607617,21.0828995309025,-16.8510851057225));
#102932=CARTESIAN_POINT('Ctrl Pts',(-19.722684372029,21.0829487769765,-16.8510914205397));
#102933=CARTESIAN_POINT('Ctrl Pts',(-19.7224825634121,21.0830553509191,
-16.8511050878986));
#102934=CARTESIAN_POINT('Ctrl Pts',(-19.7223739885994,21.0831126765595,
-16.8511124403841));
#102935=CARTESIAN_POINT('Ctrl Pts',(-19.7221390309196,21.0832367040508,
-16.8511283498257));
#102936=CARTESIAN_POINT('Ctrl Pts',(-19.7220126465365,21.0833034024179,
-16.8511369066456));
#102937=CARTESIAN_POINT('Ctrl Pts',(-19.7217267223079,21.0834542596749,
-16.8511562630028));
#102938=CARTESIAN_POINT('Ctrl Pts',(-19.7215671784302,21.0835384109874,
-16.8511670622719));
#102939=CARTESIAN_POINT('Ctrl Pts',(-19.7156957196511,21.08663434892,-16.8515644384269));
#102940=CARTESIAN_POINT('Ctrl Pts',(-19.7099700173434,21.0896200316995,
-16.8519500877194));
#102941=CARTESIAN_POINT('Ctrl Pts',(-19.696713170044,21.0964558843378,-16.8528387449199));
#102942=CARTESIAN_POINT('Ctrl Pts',(-19.6891724004307,21.1002872275498,
-16.8533410856229));
#102943=CARTESIAN_POINT('Ctrl Pts',(-19.6688198113224,21.1104750486426,
-16.8546886005082));
#102944=CARTESIAN_POINT('Ctrl Pts',(-19.6559660662701,21.1167471310882,
-16.8555308270215));
#102945=CARTESIAN_POINT('Ctrl Pts',(-19.5375058173773,21.1730716635396,
-16.8632150173504));
#102946=CARTESIAN_POINT('Ctrl Pts',(-19.4279816947245,21.2144324256188,
-16.8697401399791));
#102947=CARTESIAN_POINT('Ctrl Pts',(-19.1589186075763,21.2913083686041,
-16.8850590384475));
#102948=CARTESIAN_POINT('Ctrl Pts',(-18.9976226529485,21.3178293447792,
-16.893669114829));
#102949=CARTESIAN_POINT('Ctrl Pts',(-18.8026638245846,21.3271323320097,
-16.9048789539896));
#102950=CARTESIAN_POINT('Ctrl Pts',(-18.7703950822212,21.3279331376575,
-16.9067618072207));
#102951=CARTESIAN_POINT('Ctrl Pts',(-18.7308990050844,21.3280100532676,
-16.909113528753));
#102952=CARTESIAN_POINT('Ctrl Pts',(-18.7236754149912,21.3279871471808,
-16.9095455751668));
#102953=CARTESIAN_POINT('Ctrl Pts',(-18.7123461453106,21.3278932357209,
-16.9102264093285));
#102954=CARTESIAN_POINT('Ctrl Pts',(-18.7082402359922,21.3278472535267,
-16.9104738190418));
#102955=CARTESIAN_POINT('Ctrl Pts',(-18.7005624300027,21.3277389284762,
-16.9109377461045));
#102956=CARTESIAN_POINT('Ctrl Pts',(-18.6969905485386,21.3276794897332,
-16.9111540993871));
#102957=CARTESIAN_POINT('Ctrl Pts',(-18.6888328761138,21.3275230851003,
-16.9116494082892));
#102958=CARTESIAN_POINT('Ctrl Pts',(-18.6842472546522,21.3274202565319,
-16.9119286875966));
#102959=CARTESIAN_POINT('Ctrl Pts',(-18.6701379119595,21.3270579866315,
-16.9127905463215));
#102960=CARTESIAN_POINT('Ctrl Pts',(-18.6606157325954,21.3267491605994,
-16.9133757823429));
#102961=CARTESIAN_POINT('Ctrl Pts',(-18.531580303092,21.3216921253335,-16.9213519302441));
#102962=CARTESIAN_POINT('Ctrl Pts',(-18.4126898090621,21.3068883823168,
-16.9292197319498));
#102963=CARTESIAN_POINT('Ctrl Pts',(-18.1890914981612,21.2595698134871,
-16.9443184106419));
#102964=CARTESIAN_POINT('Ctrl Pts',(-18.0843748731905,21.2288092643061,
-16.9515213934213));
#102965=CARTESIAN_POINT('Ctrl Pts',(-17.9123350918901,21.1634821687294,
-16.9633453241773));
#102966=CARTESIAN_POINT('Ctrl Pts',(-17.8436435457359,21.1331309454483,
-16.9680664510751));
#102967=CARTESIAN_POINT('Ctrl Pts',(-17.759926684429,21.0906871888177,-16.9738164513622));
#102968=CARTESIAN_POINT('Ctrl Pts',(-17.7432648938693,21.0819587748617,
-16.9749608276412));
#102969=CARTESIAN_POINT('Ctrl Pts',(-17.7191971258834,21.0689389939885,
-16.9766142771739));
#102970=CARTESIAN_POINT('Ctrl Pts',(-17.7116977028387,21.064823129447,-16.9771295464027));
#102971=CARTESIAN_POINT('Ctrl Pts',(-17.6985885393089,21.0575247627869,
-16.9780304226833));
#102972=CARTESIAN_POINT('Ctrl Pts',(-17.6929680489618,21.0543618936229,
-16.9784167256709));
#102973=CARTESIAN_POINT('Ctrl Pts',(-17.6820792410735,21.0481686512974,
-16.979165272827));
#102974=CARTESIAN_POINT('Ctrl Pts',(-17.6768093527798,21.0451411813123,
-16.9795276165287));
#102975=CARTESIAN_POINT('Ctrl Pts',(-17.6642374714318,21.0378466431114,
-16.9803922280677));
#102976=CARTESIAN_POINT('Ctrl Pts',(-17.6569478312777,21.0335584089353,
-16.9808937253888));
#102977=CARTESIAN_POINT('Ctrl Pts',(-17.6307063686194,21.0179090732608,
-16.9826998081923));
#102978=CARTESIAN_POINT('Ctrl Pts',(-17.6119065862974,21.006294867484,-16.9839951696617));
#102979=CARTESIAN_POINT('Ctrl Pts',(-17.4368620860328,20.8943311627244,
-16.9960803616487));
#102980=CARTESIAN_POINT('Ctrl Pts',(-17.2942802230183,20.7741326048051,
-17.0060124385862));
#102981=CARTESIAN_POINT('Ctrl Pts',(-17.1152684613226,20.5776780387714,
-17.0205016160832));
#102982=CARTESIAN_POINT('Ctrl Pts',(-17.0647424197582,20.5154837231388,
-17.0249052943029));
#102983=CARTESIAN_POINT('Ctrl Pts',(-16.9967780191285,20.4213906871449,
-17.031544840602));
#102984=CARTESIAN_POINT('Ctrl Pts',(-16.9764416504457,20.3916668142064,
-17.0336395237962));
#102985=CARTESIAN_POINT('Ctrl Pts',(-16.9528178017769,20.3551742457764,
-17.0362265788814));
#102986=CARTESIAN_POINT('Ctrl Pts',(-16.9487942786771,20.3488863109973,
-17.0366728863048));
#102987=CARTESIAN_POINT('Ctrl Pts',(-16.9425810575411,20.3390622635854,
-17.0373712331894));
#102988=CARTESIAN_POINT('Ctrl Pts',(-16.9403683357703,20.3355406841529,
-17.0376217752691));
#102989=CARTESIAN_POINT('Ctrl Pts',(-16.9362777634657,20.3289876905151,
-17.0380884186271));
#102990=CARTESIAN_POINT('Ctrl Pts',(-16.9343971895342,20.3259580439778,
-17.03830433641));
#102991=CARTESIAN_POINT('Ctrl Pts',(-16.930155003285,20.3190850941592,-17.0387945488531));
#102992=CARTESIAN_POINT('Ctrl Pts',(-16.9277980269234,20.3152390047697,
-17.0390691411588));
#102993=CARTESIAN_POINT('Ctrl Pts',(-16.9217436399011,20.3052882723997,
-17.0397802121716));
#102994=CARTESIAN_POINT('Ctrl Pts',(-16.91806481064,20.2991724691257,-17.0402178582158));
#102995=CARTESIAN_POINT('Ctrl Pts',(-16.8956528701362,20.2614839826538,
-17.042918049991));
#102996=CARTESIAN_POINT('Ctrl Pts',(-16.8777139434229,20.229449050776,-17.0452268991277));
#102997=CARTESIAN_POINT('Ctrl Pts',(-16.7812828198082,20.0462254354891,
-17.0584408825197));
#102998=CARTESIAN_POINT('Ctrl Pts',(-16.7204310367164,19.8864620716192,
-17.069934485297));
#102999=CARTESIAN_POINT('Ctrl Pts',(-16.6563717005341,19.6284539752063,
-17.0872114878343));
#103000=CARTESIAN_POINT('Ctrl Pts',(-16.6396560788146,19.5343186919745,
-17.0932786793386));
#103001=CARTESIAN_POINT('Ctrl Pts',(-16.6270441989163,19.4180854513586,
-17.1004603678851));
#103002=CARTESIAN_POINT('Ctrl Pts',(-16.6250580935117,19.3967719563002,
-17.1017650354998));
#103003=CARTESIAN_POINT('Ctrl Pts',(-16.6226955365492,19.3664467011526,
-17.1036045885643));
#103004=CARTESIAN_POINT('Ctrl Pts',(-16.6220529349184,19.3574575450612,
-17.1041477933856));
#103005=CARTESIAN_POINT('Ctrl Pts',(-16.6210439417596,19.341951495327,-17.1050812903387));
#103006=CARTESIAN_POINT('Ctrl Pts',(-16.6206502556039,19.3354365602431,
-17.1054724341047));
#103007=CARTESIAN_POINT('Ctrl Pts',(-16.6199544833816,19.3229648433948,
-17.1062192021889));
#103008=CARTESIAN_POINT('Ctrl Pts',(-16.6196474299979,19.3170084116352,
-17.1065749786924));
#103009=CARTESIAN_POINT('Ctrl Pts',(-16.6189150554614,19.301529217575,-17.1074973131409));
#103010=CARTESIAN_POINT('Ctrl Pts',(-16.6185288681592,19.2920046709398,
-17.1080626404137));
#103011=CARTESIAN_POINT('Ctrl Pts',(-16.6174336282252,19.2595847652786,
-17.1099796902197));
#103012=CARTESIAN_POINT('Ctrl Pts',(-16.6170318197903,19.236680143847,-17.1113218040137));
#103013=CARTESIAN_POINT('Ctrl Pts',(-16.6167704938624,19.0371634066197,
-17.1229164096785));
#103014=CARTESIAN_POINT('Ctrl Pts',(-16.6386380699323,18.86122154183,-17.1324066911915));
#103015=CARTESIAN_POINT('Ctrl Pts',(-16.7033215799155,18.606461136644,-17.1467108838563));
#103016=CARTESIAN_POINT('Ctrl Pts',(-16.7296217467567,18.5242776749342,
-17.1514331796244));
#103017=CARTESIAN_POINT('Ctrl Pts',(-16.7744878690877,18.4088674171645,
-17.1585043311072));
#103018=CARTESIAN_POINT('Ctrl Pts',(-16.7890513907631,18.3741732642092,
-17.1606900626565));
#103019=CARTESIAN_POINT('Ctrl Pts',(-16.8076413207388,18.3329974966708,
-17.1633780849125));
#103020=CARTESIAN_POINT('Ctrl Pts',(-16.8107890696741,18.3261238105902,
-17.1638300088621));
#103021=CARTESIAN_POINT('Ctrl Pts',(-16.8157341398824,18.315476376396,-17.1645352467976));
#103022=CARTESIAN_POINT('Ctrl Pts',(-16.8175059704469,18.3116907625741,
-17.1647870152137));
#103023=CARTESIAN_POINT('Ctrl Pts',(-16.8208093462708,18.3046870162201,
-17.1652547600238));
#103024=CARTESIAN_POINT('Ctrl Pts',(-16.8223378114088,18.3014674946924,
-17.165470545438));
#103025=CARTESIAN_POINT('Ctrl Pts',(-16.8258074075702,18.2942066041377,
-17.1659589357799));
#103026=CARTESIAN_POINT('Ctrl Pts',(-16.82775324015,18.2901675558462,-17.1662318288778));
#103027=CARTESIAN_POINT('Ctrl Pts',(-16.833521780004,18.2782901908661,-17.1670378210301));
#103028=CARTESIAN_POINT('Ctrl Pts',(-16.8373800541377,18.2704693903541,
-17.1675730571942));
#103029=CARTESIAN_POINT('Ctrl Pts',(-16.8651906123301,18.2149638428839,
-17.171402806243));
#103030=CARTESIAN_POINT('Ctrl Pts',(-16.8908880166505,18.1681799131341,
-17.1747944450502));
#103031=CARTESIAN_POINT('Ctrl Pts',(-16.92737026789,18.1073299326637,-17.1793798262357));
#103032=CARTESIAN_POINT('Ctrl Pts',(-16.9366057134555,18.0923524411188,
-17.1805230519075));
#103033=CARTESIAN_POINT('Ctrl Pts',(-16.9719970248176,18.0365268713673,
-17.1848350321887));
#103034=CARTESIAN_POINT('Ctrl Pts',(-16.9993670063192,17.9964672694417,
-17.1880325456117));
#103035=CARTESIAN_POINT('Ctrl Pts',(-17.092860645783,17.8692417428287,-17.198461929987));
#103036=CARTESIAN_POINT('Ctrl Pts',(-17.16437244302,17.7862451443228,-17.2056947298553));
#103037=CARTESIAN_POINT('Ctrl Pts',(-17.2810732630817,17.6703088986067,
-17.2162683797988));
#103038=CARTESIAN_POINT('Ctrl Pts',(-17.3216673655765,17.6330131421397,
-17.2197576070219));
#103039=CARTESIAN_POINT('Ctrl Pts',(-17.3898211512651,17.5751366283048,
-17.2253153036747));
#103040=CARTESIAN_POINT('Ctrl Pts',(-17.416505748954,17.5535698014598,-17.2274222140389));
#103041=CARTESIAN_POINT('Ctrl Pts',(-17.4522728821646,17.5260722807138,
-17.2301587913689));
#103042=CARTESIAN_POINT('Ctrl Pts',(-17.4608922230727,17.5195502020674,
-17.2308118006939));
#103043=CARTESIAN_POINT('Ctrl Pts',(-17.47509371396,17.508974281704,-17.2318773062803));
#103044=CARTESIAN_POINT('Ctrl Pts',(-17.4806463190806,17.5048812658405,
-17.2322913320175));
#103045=CARTESIAN_POINT('Ctrl Pts',(-17.4914348492334,17.4970097621399,
-17.2330908478878));
#103046=CARTESIAN_POINT('Ctrl Pts',(-17.4966682435219,17.4932279501588,
-17.2334764643715));
#103047=CARTESIAN_POINT('Ctrl Pts',(-17.5087941182849,17.4845495872985,
-17.2343648817411));
#103048=CARTESIAN_POINT('Ctrl Pts',(-17.5156988228576,17.479670243702,-17.2348670165765));
#103049=CARTESIAN_POINT('Ctrl Pts',(-17.5343516749213,17.4666556849718,
-17.2362136146957));
#103050=CARTESIAN_POINT('Ctrl Pts',(-17.5461533940615,17.4585977491154,
-17.2370551366544));
#103051=CARTESIAN_POINT('Ctrl Pts',(-17.6551778851291,17.3857658766104,
-17.2447362189286));
#103052=CARTESIAN_POINT('Ctrl Pts',(-17.7575303306774,17.3290199236885,
-17.2512591698624));
#103053=CARTESIAN_POINT('Ctrl Pts',(-18.0124241071135,17.2141266389694,
-17.2665653225836));
#103054=CARTESIAN_POINT('Ctrl Pts',(-18.1679915624739,17.164589097064,-17.2751654339514));
#103055=CARTESIAN_POINT('Ctrl Pts',(-18.359578288624,17.1271204164737,-17.286374450996));
#103056=CARTESIAN_POINT('Ctrl Pts',(-18.3916189142075,17.1216171563284,
-17.2882704403549));
#103057=CARTESIAN_POINT('Ctrl Pts',(-18.4309328911563,17.1157931513323,
-17.2906367771272));
#103058=CARTESIAN_POINT('Ctrl Pts',(-18.438099569571,17.1147690148756,-17.2910697605058));
#103059=CARTESIAN_POINT('Ctrl Pts',(-18.4493425258526,17.1132211718275,
-17.2917517458983));
#103060=CARTESIAN_POINT('Ctrl Pts',(-18.4534153935769,17.1126725309201,
-17.2919993621683));
#103061=CARTESIAN_POINT('Ctrl Pts',(-18.4610311400588,17.1116692113184,
-17.2924634637215));
#103062=CARTESIAN_POINT('Ctrl Pts',(-18.4645735807839,17.1112116385749,
-17.2926797836414));
#103063=CARTESIAN_POINT('Ctrl Pts',(-18.4726624110747,17.1101876202075,
-17.2931747353383));
#103064=CARTESIAN_POINT('Ctrl Pts',(-18.4772094761604,17.1096269687584,
-17.2934536889974));
#103065=CARTESIAN_POINT('Ctrl Pts',(-18.4911909812095,17.1079491119574,
-17.2943135670052));
#103066=CARTESIAN_POINT('Ctrl Pts',(-18.5006309991433,17.1068806690185,
-17.294897130639));
#103067=CARTESIAN_POINT('Ctrl Pts',(-18.5854881532004,17.0978544031714,
-17.3001677509269));
#103068=CARTESIAN_POINT('Ctrl Pts',(-18.6612672861743,17.0938917141039,
-17.3050495259045));
#103069=CARTESIAN_POINT('Ctrl Pts',(-18.9220107228818,17.0942718487392,
-17.3221024429291));
#103070=CARTESIAN_POINT('Ctrl Pts',(-19.1061424033332,17.1187724827416,
-17.3344993698907));
#103071=CARTESIAN_POINT('Ctrl Pts',(-19.3361780933514,17.1807519209795,
-17.349526425177));
#103072=CARTESIAN_POINT('Ctrl Pts',(-19.3870669939627,17.1965447340662,
-17.3528279642546));
#103073=CARTESIAN_POINT('Ctrl Pts',(-19.4491380982266,17.2184077771642,
-17.3568295944672));
#103074=CARTESIAN_POINT('Ctrl Pts',(-19.4609293340424,17.222679095327,-17.3575886440234));
#103075=CARTESIAN_POINT('Ctrl Pts',(-19.4795055394213,17.2295955727872,
-17.3587828706293));
#103076=CARTESIAN_POINT('Ctrl Pts',(-19.4863158701772,17.2321713447019,
-17.3592203514209));
#103077=CARTESIAN_POINT('Ctrl Pts',(-19.4990579924253,17.2370659007478,
-17.3600382827464));
#103078=CARTESIAN_POINT('Ctrl Pts',(-19.5049928552492,17.2393764105466,
-17.3604190051709));
#103079=CARTESIAN_POINT('Ctrl Pts',(-19.5182500967761,17.2446066198789,
-17.3612689560568));
#103080=CARTESIAN_POINT('Ctrl Pts',(-19.5255668007745,17.247540516802,-17.361737700704));
#103081=CARTESIAN_POINT('Ctrl Pts',(-19.5440621451908,17.2550770817718,
-17.362921827671));
#103082=CARTESIAN_POINT('Ctrl Pts',(-19.5552181562344,17.2597347976033,
-17.3636353444181));
#103083=CARTESIAN_POINT('Ctrl Pts',(-19.618639505344,17.2868539377761,-17.3676884237337));
#103084=CARTESIAN_POINT('Ctrl Pts',(-19.6700252934956,17.3113203944047,
-17.3709588771089));
#103085=CARTESIAN_POINT('Ctrl Pts',(-19.7441244366506,17.3503392135024,
-17.3756896458241));
#103086=CARTESIAN_POINT('Ctrl Pts',(-19.7676426166676,17.3633006331428,
-17.377193573104));
#103087=CARTESIAN_POINT('Ctrl Pts',(-19.8912833375688,17.4345416336196,
-17.3851309615017));
#103088=CARTESIAN_POINT('Ctrl Pts',(-19.9867413041996,17.5005178870648,
-17.3913558622935));
#103089=CARTESIAN_POINT('Ctrl Pts',(-20.1382147131518,17.6247226157745,
-17.4020347573932));
#103090=CARTESIAN_POINT('Ctrl Pts',(-20.1971729278717,17.6789367236937,
-17.4064365656863));
#103091=CARTESIAN_POINT('Ctrl Pts',(-20.2779937140936,17.7621837456945,
-17.4130735689769));
#103092=CARTESIAN_POINT('Ctrl Pts',(-20.3024069513658,17.7886482801445,
-17.4151677035097));
#103093=CARTESIAN_POINT('Ctrl Pts',(-20.3310516861282,17.8213343455992,
-17.4177541498842));
#103094=CARTESIAN_POINT('Ctrl Pts',(-20.3359416236859,17.8269740790997,
-17.4182004225804));
#103095=CARTESIAN_POINT('Ctrl Pts',(-20.3435094062188,17.8357960994264,
-17.418898726846));
#103096=CARTESIAN_POINT('Ctrl Pts',(-20.3462079277635,17.8389606806536,
-17.4191492613297));
#103097=CARTESIAN_POINT('Ctrl Pts',(-20.3512028449127,17.8448533481459,
-17.4196158979282));
#103098=CARTESIAN_POINT('Ctrl Pts',(-20.3535016791178,17.8475792921132,
-17.4198318165941));
#103099=CARTESIAN_POINT('Ctrl Pts',(-20.3586930694697,17.8537668661355,
-17.42032204061));
#103100=CARTESIAN_POINT('Ctrl Pts',(-20.361581440374,17.8572319239539,-17.4205966436654));
#103101=CARTESIAN_POINT('Ctrl Pts',(-20.3701034444459,17.8675221104456,
-17.42141228901));
#103102=CARTESIAN_POINT('Ctrl Pts',(-20.375705297689,17.8743732645519,-17.4219555439972));
#103103=CARTESIAN_POINT('Ctrl Pts',(-20.4168969112017,17.9254008472913,
-17.4260019210848));
#103104=CARTESIAN_POINT('Ctrl Pts',(-20.4507379835476,17.9709529555637,
-17.4296147387959));
#103105=CARTESIAN_POINT('Ctrl Pts',(-20.5175955942822,18.0689371151353,
-17.4372974290447));
#103106=CARTESIAN_POINT('Ctrl Pts',(-20.5502244118431,18.1215739265789,
-17.4413750935863));
#103107=CARTESIAN_POINT('Ctrl Pts',(-20.6341053691248,18.2711590612222,
-17.452703249606));
#103108=CARTESIAN_POINT('Ctrl Pts',(-20.6802112962647,18.3707819009973,
-17.4599518298351));
#103109=CARTESIAN_POINT('Ctrl Pts',(-20.7198023055324,18.4773144540793,
-17.4672585983927));
#103110=CARTESIAN_POINT('Ctrl Pts',(-20.7211968892606,18.4811001446346,
-17.4675177024312));
#103111=CARTESIAN_POINT('Ctrl Pts',(-20.7225806135343,18.4848897167264,
-17.4677765237272));
#103112=CARTESIAN_POINT('',(-20.8509993557841,19.2126515476976,-16.4878149913274));
#103113=CARTESIAN_POINT('Ctrl Pts',(-20.7225806138883,18.484889717696,-17.2426990599955));
#103114=CARTESIAN_POINT('Ctrl Pts',(-20.7071867113841,18.4427308103813,
-17.239882851258));
#103115=CARTESIAN_POINT('Ctrl Pts',(-20.6904549548032,18.4010691626674,
-17.2371086158738));
#103116=CARTESIAN_POINT('Ctrl Pts',(-20.6673796328444,18.3485101301596,
-17.2336176480217));
#103117=CARTESIAN_POINT('Ctrl Pts',(-20.6622477660772,18.3370971773503,
-17.2328601224428));
#103118=CARTESIAN_POINT('Ctrl Pts',(-20.6539422346179,18.3190556029706,
-17.2316632936934));
#103119=CARTESIAN_POINT('Ctrl Pts',(-20.6508347897754,18.3123969828176,
-17.2312217238274));
#103120=CARTESIAN_POINT('Ctrl Pts',(-20.6449719435814,18.300002900346,-17.2304000269476));
#103121=CARTESIAN_POINT('Ctrl Pts',(-20.6422252387044,18.2942634378015,
-17.2300196046811));
#103122=CARTESIAN_POINT('Ctrl Pts',(-20.6360566868268,18.2815215977503,
-17.2291752107988));
#103123=CARTESIAN_POINT('Ctrl Pts',(-20.6326219525082,18.2745255347363,
-17.228711693585));
#103124=CARTESIAN_POINT('Ctrl Pts',(-20.6224963106263,18.2541857537887,
-17.227364305645));
#103125=CARTESIAN_POINT('Ctrl Pts',(-20.6157027256542,18.2408934665018,
-17.2264840324975));
#103126=CARTESIAN_POINT('Ctrl Pts',(-20.5587597755292,18.132328387959,-17.2192940048285));
#103127=CARTESIAN_POINT('Ctrl Pts',(-20.5015469952183,18.0409304560815,
-17.2132500513549));
#103128=CARTESIAN_POINT('Ctrl Pts',(-20.3582443594567,17.846669251552,-17.1999840335387));
#103129=CARTESIAN_POINT('Ctrl Pts',(-20.2688562436721,17.7468341966682,
-17.192865009603));
#103130=CARTESIAN_POINT('Ctrl Pts',(-20.1586015668276,17.6449640266721,
-17.1845188886493));
#103131=CARTESIAN_POINT('Ctrl Pts',(-20.1464197126941,17.6339683485899,
-17.1836017627802));
#103132=CARTESIAN_POINT('Ctrl Pts',(-20.0943089420233,17.5880198594671,
-17.1796936555183));
#103133=CARTESIAN_POINT('Ctrl Pts',(-20.053204350568,17.5544361373716,-17.1766480658313));
#103134=CARTESIAN_POINT('Ctrl Pts',(-20.0039431423795,17.5171850233622,
-17.1729829188183));
#103135=CARTESIAN_POINT('Ctrl Pts',(-19.996968451099,17.5119780914886,-17.1724636408047));
#103136=CARTESIAN_POINT('Ctrl Pts',(-19.9863557939277,17.5041567050613,
-17.1716726575752));
#103137=CARTESIAN_POINT('Ctrl Pts',(-19.9827412141084,17.5015104716903,
-17.1714031071031));
#103138=CARTESIAN_POINT('Ctrl Pts',(-19.9762361175234,17.4967797315891,
-17.1709176823085));
#103139=CARTESIAN_POINT('Ctrl Pts',(-19.9733487146159,17.4946910349267,
-17.1707021028946));
#103140=CARTESIAN_POINT('Ctrl Pts',(-19.9670609884658,17.4901667446976,
-17.1702323873001));
#103141=CARTESIAN_POINT('Ctrl Pts',(-19.9636587615153,17.4877339661674,
-17.1699780688898));
#103142=CARTESIAN_POINT('Ctrl Pts',(-19.9540761433167,17.4809246965056,
-17.1692613665436));
#103143=CARTESIAN_POINT('Ctrl Pts',(-19.9478795178131,17.4765713149553,
-17.1687974480133));
#103144=CARTESIAN_POINT('Ctrl Pts',(-19.9105751044534,17.4506612792974,
-17.166002506873));
#103145=CARTESIAN_POINT('Ctrl Pts',(-19.8789192103176,17.429910170921,-17.1636221473655));
#103146=CARTESIAN_POINT('Ctrl Pts',(-19.7726318910349,17.364241070351,-17.1556453005459));
#103147=CARTESIAN_POINT('Ctrl Pts',(-19.6957872426308,17.3230810053705,
-17.1499056945703));
#103148=CARTESIAN_POINT('Ctrl Pts',(-19.4572798279054,17.2136790136048,
-17.1325684497204));
#103149=CARTESIAN_POINT('Ctrl Pts',(-19.2894316466971,17.160647855784,-17.1210588431207));
#103150=CARTESIAN_POINT('Ctrl Pts',(-19.0943199638128,17.1247623385175,
-17.1088478016649));
#103151=CARTESIAN_POINT('Ctrl Pts',(-19.0716312042711,17.1209705045342,
-17.1074436467772));
#103152=CARTESIAN_POINT('Ctrl Pts',(-19.0394428363058,17.1161289218101,
-17.1054732096206));
#103153=CARTESIAN_POINT('Ctrl Pts',(-19.0299916262415,17.1147726453569,
-17.1048972686811));
#103154=CARTESIAN_POINT('Ctrl Pts',(-19.0146192467303,17.1126727031556,
-17.1039646760883));
#103155=CARTESIAN_POINT('Ctrl Pts',(-19.00870361759,17.111890062447,-17.1036067962195));
#103156=CARTESIAN_POINT('Ctrl Pts',(-18.9963132670565,17.1103040877661,
-17.1028592798134));
#103157=CARTESIAN_POINT('Ctrl Pts',(-18.9898379734459,17.1095056510752,
-17.1024698016247));
#103158=CARTESIAN_POINT('Ctrl Pts',(-18.9744234451177,17.1076772631884,
-17.1015453993111));
#103159=CARTESIAN_POINT('Ctrl Pts',(-18.9654810848497,17.106674340955,-17.1010113324702));
#103160=CARTESIAN_POINT('Ctrl Pts',(-18.9353274390045,17.1034870247805,
-17.0992176712833));
#103161=CARTESIAN_POINT('Ctrl Pts',(-18.9140891868463,17.1015660446221,
-17.0979663603395));
#103162=CARTESIAN_POINT('Ctrl Pts',(-18.798277175956,17.0928528555167,-17.0912031111308));
#103163=CARTESIAN_POINT('Ctrl Pts',(-18.7033525915127,17.0920987165368,
-17.0858843512766));
#103164=CARTESIAN_POINT('Ctrl Pts',(-18.4395270354852,17.1077428381018,
-17.0713425025402));
#103165=CARTESIAN_POINT('Ctrl Pts',(-18.2722026975441,17.1380463670778,
-17.0624253753528));
#103166=CARTESIAN_POINT('Ctrl Pts',(-18.0737616979252,17.1992256097341,
-17.050582336029));
#103167=CARTESIAN_POINT('Ctrl Pts',(-18.0375393841443,17.2114768031053,
-17.0483639154203));
#103168=CARTESIAN_POINT('Ctrl Pts',(-17.9948887057446,17.227201685988,-17.0456619415993));
#103169=CARTESIAN_POINT('Ctrl Pts',(-17.9881191384273,17.2297370207558,
-17.0452303515146));
#103170=CARTESIAN_POINT('Ctrl Pts',(-17.9771205158353,17.233920576392,-17.0445244842911));
#103171=CARTESIAN_POINT('Ctrl Pts',(-17.9728834784367,17.235547838968,-17.0442514307876));
#103172=CARTESIAN_POINT('Ctrl Pts',(-17.9653249718972,17.2384786610419,
-17.0437622510861));
#103173=CARTESIAN_POINT('Ctrl Pts',(-17.9620015356182,17.2397770034293,
-17.0435464397254));
#103174=CARTESIAN_POINT('Ctrl Pts',(-17.9548299797033,17.2425995808095,
-17.0430791717802));
#103175=CARTESIAN_POINT('Ctrl Pts',(-17.9509830972108,17.2441266792019,
-17.0428275489283));
#103176=CARTESIAN_POINT('Ctrl Pts',(-17.9402960506349,17.2484054416186,
-17.0421258453779));
#103177=CARTESIAN_POINT('Ctrl Pts',(-17.9334658233721,17.2511815420306,
-17.0416743294713));
#103178=CARTESIAN_POINT('Ctrl Pts',(-17.894731808093,17.2671609928011,-17.0390970123892));
#103179=CARTESIAN_POINT('Ctrl Pts',(-17.8631422551203,17.2811068283179,
-17.0369302217592));
#103180=CARTESIAN_POINT('Ctrl Pts',(-17.7643243603082,17.3276520781118,
-17.0299765195953));
#103181=CARTESIAN_POINT('Ctrl Pts',(-17.6984756342572,17.3630395037646,
-17.0250816208564));
#103182=CARTESIAN_POINT('Ctrl Pts',(-17.4687841841863,17.5026137963652,
-17.0073544895979));
#103183=CARTESIAN_POINT('Ctrl Pts',(-17.3175337167249,17.6257525923294,
-16.9945292851593));
#103184=CARTESIAN_POINT('Ctrl Pts',(-17.1707664458559,17.783261773556,-16.9813025167347));
#103185=CARTESIAN_POINT('Ctrl Pts',(-17.1565918516148,17.7989379715176,
-16.9800140347842));
#103186=CARTESIAN_POINT('Ctrl Pts',(-17.1371797250755,17.8210637037834,
-16.9782332452673));
#103187=CARTESIAN_POINT('Ctrl Pts',(-17.1317421870163,17.8273353723708,
-16.977732599134));
#103188=CARTESIAN_POINT('Ctrl Pts',(-17.122414129,17.8382230989188,-16.9768705062795));
#103189=CARTESIAN_POINT('Ctrl Pts',(-17.118506237229,17.8428240817167,-16.9765083432027));
#103190=CARTESIAN_POINT('Ctrl Pts',(-17.1104489428885,17.8523930437213,
-16.9757595252879));
#103191=CARTESIAN_POINT('Ctrl Pts',(-17.1063025336129,17.8573634697416,
-16.9753729954568));
#103192=CARTESIAN_POINT('Ctrl Pts',(-17.0966354339348,17.8690603595251,
-16.9744690045393));
#103193=CARTESIAN_POINT('Ctrl Pts',(-17.0911332646778,17.8758020317935,
-16.9739522991281));
#103194=CARTESIAN_POINT('Ctrl Pts',(-17.0733610097538,17.8978541216328,
-16.9722759722131));
#103195=CARTESIAN_POINT('Ctrl Pts',(-17.0612619401687,17.9133015083381,
-16.9711232061933));
#103196=CARTESIAN_POINT('Ctrl Pts',(-17.0002276133366,17.9934987853206,
-16.9652438486283));
#103197=CARTESIAN_POINT('Ctrl Pts',(-16.9548276551289,18.0608592497496,
-16.9606564668553));
#103198=CARTESIAN_POINT('Ctrl Pts',(-16.8273632954993,18.2756643202835,
-16.9468136257089));
#103199=CARTESIAN_POINT('Ctrl Pts',(-16.7589599285342,18.4304070669432,
-16.9379421871519));
#103200=CARTESIAN_POINT('Ctrl Pts',(-16.6938873449351,18.643085417118,-16.9254391539659));
#103201=CARTESIAN_POINT('Ctrl Pts',(-16.6801083694984,18.6951368935616,
-16.9223514123593));
#103202=CARTESIAN_POINT('Ctrl Pts',(-16.666416362408,18.7561777806655,-16.9186391868716));
#103203=CARTESIAN_POINT('Ctrl Pts',(-16.6645567538077,18.7647153436713,
-16.9181179175073));
#103204=CARTESIAN_POINT('Ctrl Pts',(-16.6618222983134,18.7776540573983,
-16.9173244912749));
#103205=CARTESIAN_POINT('Ctrl Pts',(-16.6609084785371,18.7820470001002,
-16.9170545091197));
#103206=CARTESIAN_POINT('Ctrl Pts',(-16.6592938471777,18.7899345856513,
-16.9165686253111));
#103207=CARTESIAN_POINT('Ctrl Pts',(-16.658587889457,18.7934281201549,-16.9163530210267));
#103208=CARTESIAN_POINT('Ctrl Pts',(-16.6570737503213,18.801019755965,-16.9158836238743));
#103209=CARTESIAN_POINT('Ctrl Pts',(-16.6562688847687,18.8051184172599,
-16.91562965081));
#103210=CARTESIAN_POINT('Ctrl Pts',(-16.6540437725974,18.8166295469774,
-16.9149148758286));
#103211=CARTESIAN_POINT('Ctrl Pts',(-16.6526510446535,18.8240471808273,
-16.9144525522565));
#103212=CARTESIAN_POINT('Ctrl Pts',(-16.6445932495909,18.8682652212819,
-16.9116868942807));
#103213=CARTESIAN_POINT('Ctrl Pts',(-16.6388650967294,18.9052271479884,
-16.9093353927574));
#103214=CARTESIAN_POINT('Ctrl Pts',(-16.6232881090554,19.0269691751384,
-16.9015022194512));
#103215=CARTESIAN_POINT('Ctrl Pts',(-16.617586258404,19.112191936991,-16.8958826046338));
#103216=CARTESIAN_POINT('Ctrl Pts',(-16.615910509217,19.3753571119182,-16.8784969082499));
#103217=CARTESIAN_POINT('Ctrl Pts',(-16.6371917536044,19.5526663831567,
-16.8668109489057));
#103218=CARTESIAN_POINT('Ctrl Pts',(-16.6859482611975,19.7473704050032,
-16.8544587546291));
#103219=CARTESIAN_POINT('Ctrl Pts',(-16.6918455597985,19.7694034763491,
-16.8530666616067));
#103220=CARTESIAN_POINT('Ctrl Pts',(-16.7007065194646,19.8004889076983,
-16.8511100590181));
#103221=CARTESIAN_POINT('Ctrl Pts',(-16.7033768078006,19.8096225907979,
-16.8505360737049));
#103222=CARTESIAN_POINT('Ctrl Pts',(-16.7078199692388,19.8244484657939,
-16.8496057825708));
#103223=CARTESIAN_POINT('Ctrl Pts',(-16.7095554395363,19.8301516453819,
-16.8492482605189));
#103224=CARTESIAN_POINT('Ctrl Pts',(-16.713242176425,19.8420859299351,-16.8485008050157));
#103225=CARTESIAN_POINT('Ctrl Pts',(-16.7151982296767,19.848315499666,-16.8481110329277));
#103226=CARTESIAN_POINT('Ctrl Pts',(-16.7199269485865,19.863135122253,-16.8471846832048));
#103227=CARTESIAN_POINT('Ctrl Pts',(-16.7227258076438,19.8717167328822,
-16.8466489726007));
#103228=CARTESIAN_POINT('Ctrl Pts',(-16.7323733050803,19.900667580712,-16.8448439076605));
#103229=CARTESIAN_POINT('Ctrl Pts',(-16.739477314475,19.9209507762255,-16.843582983214));
#103230=CARTESIAN_POINT('Ctrl Pts',(-16.8087247777823,20.1094154794984,
-16.8318925501622));
#103231=CARTESIAN_POINT('Ctrl Pts',(-16.8916862556132,20.2691692318284,
-16.8222582197732));
#103232=CARTESIAN_POINT('Ctrl Pts',(-17.0625168907625,20.5157583398618,
-16.8059327876054));
#103233=CARTESIAN_POINT('Ctrl Pts',(-17.1395800171256,20.6088792948023,
-16.7993132713628));
#103234=CARTESIAN_POINT('Ctrl Pts',(-17.2307915423774,20.7016855505723,
-16.7916011596479));
#103235=CARTESIAN_POINT('Ctrl Pts',(-17.2374895389496,20.708409599987,-16.7910354319514));
#103236=CARTESIAN_POINT('Ctrl Pts',(-17.2474861560193,20.7183110379497,
-16.7901915586537));
#103237=CARTESIAN_POINT('Ctrl Pts',(-17.2507503458532,20.7215232325391,
-16.7899160814427));
#103238=CARTESIAN_POINT('Ctrl Pts',(-17.2565788173557,20.7272217537287,
-16.7894242662379));
#103239=CARTESIAN_POINT('Ctrl Pts',(-17.2591389934707,20.7297122072974,
-16.7892082568314));
#103240=CARTESIAN_POINT('Ctrl Pts',(-17.2646594467497,20.7350551952702,
-16.7887425119715));
#103241=CARTESIAN_POINT('Ctrl Pts',(-17.2676216903343,20.7379055478104,
-16.7884926206246));
#103242=CARTESIAN_POINT('Ctrl Pts',(-17.2758275556728,20.7457555554688,
-16.787800500386));
#103243=CARTESIAN_POINT('Ctrl Pts',(-17.2810885127126,20.7507368928004,
-16.7873568982264));
#103244=CARTESIAN_POINT('Ctrl Pts',(-17.3101542708379,20.7779762056212,
-16.7849073280805));
#103245=CARTESIAN_POINT('Ctrl Pts',(-17.3344436483625,20.7997079145158,
-16.7828648986443));
#103246=CARTESIAN_POINT('Ctrl Pts',(-17.4829168238425,20.9264992702536,
-16.7704577413008));
#103247=CARTESIAN_POINT('Ctrl Pts',(-17.6183682463526,21.0175194677178,
-16.7595039646589));
#103248=CARTESIAN_POINT('Ctrl Pts',(-17.8667255663329,21.1457287814896,
-16.7412474600421));
#103249=CARTESIAN_POINT('Ctrl Pts',(-17.9748185377253,21.1906443420851,
-16.7338049997294));
#103250=CARTESIAN_POINT('Ctrl Pts',(-18.0996629589965,21.2307794421858,
-16.7257980292985));
#103251=CARTESIAN_POINT('Ctrl Pts',(-18.1132870171746,21.2350078767764,
-16.7249315812421));
#103252=CARTESIAN_POINT('Ctrl Pts',(-18.1350456189993,21.2415206245296,
-16.7235592271816));
#103253=CARTESIAN_POINT('Ctrl Pts',(-18.143152713155,21.2438944497979,-16.7230504060531));
#103254=CARTESIAN_POINT('Ctrl Pts',(-18.1574800530819,21.2479966678452,
-16.7221555389638));
#103255=CARTESIAN_POINT('Ctrl Pts',(-18.1636943625298,21.2497452404134,
-16.7217688392333));
#103256=CARTESIAN_POINT('Ctrl Pts',(-18.1765681302003,21.2533041727919,
-16.7209706722368));
#103257=CARTESIAN_POINT('Ctrl Pts',(-18.1832286444323,21.2551104518327,
-16.7205593415882));
#103258=CARTESIAN_POINT('Ctrl Pts',(-18.2003563993105,21.2596655713613,
-16.7195056745142));
#103259=CARTESIAN_POINT('Ctrl Pts',(-18.2108361826824,21.2623667986662,
-16.7188648848971));
#103260=CARTESIAN_POINT('Ctrl Pts',(-18.2547333722116,21.273323287774,-16.7161966199843));
#103261=CARTESIAN_POINT('Ctrl Pts',(-18.2883299930917,21.2808435417425,
-16.7141928453244));
#103262=CARTESIAN_POINT('Ctrl Pts',(-18.3764011492549,21.2983133654515,
-16.7090277642644));
#103263=CARTESIAN_POINT('Ctrl Pts',(-18.4311098697273,21.3069513939323,
-16.7059062700289));
#103264=CARTESIAN_POINT('Ctrl Pts',(-18.5949037264779,21.3262646694435,
-16.6967375565202));
#103265=CARTESIAN_POINT('Ctrl Pts',(-18.7045446938713,21.3306286558589,
-16.6908389834021));
#103266=CARTESIAN_POINT('Ctrl Pts',(-18.8743201135194,21.3242059362996,
-16.6815879088552));
#103267=CARTESIAN_POINT('Ctrl Pts',(-18.9344822662438,21.3193489445556,
-16.6782842403984));
#103268=CARTESIAN_POINT('Ctrl Pts',(-19.0521688847756,21.3047649593261,
-16.6716413980506));
#103269=CARTESIAN_POINT('Ctrl Pts',(-19.1096601591585,21.2952171903307,
-16.6683100094204));
#103270=CARTESIAN_POINT('Ctrl Pts',(-19.1753962908968,21.2814921207549,
-16.66432638293));
#103271=CARTESIAN_POINT('Ctrl Pts',(-19.1841020488695,21.2796170373071,
-16.6637952399934));
#103272=CARTESIAN_POINT('Ctrl Pts',(-19.1972109821879,21.2767069111776,
-16.662989710264));
#103273=CARTESIAN_POINT('Ctrl Pts',(-19.2016232210985,21.2757125657397,
-16.6627175984626));
#103274=CARTESIAN_POINT('Ctrl Pts',(-19.2095092346167,21.2739087934581,
-16.6622294347398));
#103275=CARTESIAN_POINT('Ctrl Pts',(-19.2129841798264,21.2731047203139,
-16.662013692306));
#103276=CARTESIAN_POINT('Ctrl Pts',(-19.2204981936619,21.2713460225014,
-16.6615457961641));
#103277=CARTESIAN_POINT('Ctrl Pts',(-19.2245364361732,21.2703883142762,
-16.6612934720148));
#103278=CARTESIAN_POINT('Ctrl Pts',(-19.2357911658836,21.267684164843,-16.6605878759697));
#103279=CARTESIAN_POINT('Ctrl Pts',(-19.2430012379439,21.2659116438646,
-16.6601331433608));
#103280=CARTESIAN_POINT('Ctrl Pts',(-19.2844887482649,21.2554806318736,
-16.6575015298148));
#103281=CARTESIAN_POINT('Ctrl Pts',(-19.3185521936582,21.246003024397,-16.6552816515936));
#103282=CARTESIAN_POINT('Ctrl Pts',(-19.4266352137431,21.2129932221847,
-16.6480819461551));
#103283=CARTESIAN_POINT('Ctrl Pts',(-19.4996010915503,21.1862401713975,
-16.6429860613657));
#103284=CARTESIAN_POINT('Ctrl Pts',(-19.7409861171084,21.0823485349081,
-16.6256430936995));
#103285=CARTESIAN_POINT('Ctrl Pts',(-19.9007479225477,20.987145413116,-16.6134216776107));
#103286=CARTESIAN_POINT('Ctrl Pts',(-20.0655029094118,20.8570256499575,
-16.6004774142145));
#103287=CARTESIAN_POINT('Ctrl Pts',(-20.084638660179,20.8413606131972,-16.5989662136807));
#103288=CARTESIAN_POINT('Ctrl Pts',(-20.1109989140703,20.8189986909739,
-16.5968726456078));
#103289=CARTESIAN_POINT('Ctrl Pts',(-20.1184572411664,20.8125817031984,
-16.5962789308566));
#103290=CARTESIAN_POINT('Ctrl Pts',(-20.130407174693,20.8021543771936,-16.5953253637832));
#103291=CARTESIAN_POINT('Ctrl Pts',(-20.1349268158889,20.7981765205181,
-16.5949641726114));
#103292=CARTESIAN_POINT('Ctrl Pts',(-20.1439814152561,20.7901385175708,
-16.5942394507293));
#103293=CARTESIAN_POINT('Ctrl Pts',(-20.1485159557699,20.7860779857233,
-16.5938759411892));
#103294=CARTESIAN_POINT('Ctrl Pts',(-20.1592298922481,20.7764004242386,
-16.5930156685046));
#103295=CARTESIAN_POINT('Ctrl Pts',(-20.1653937195489,20.7707662506442,
-16.5925196350218));
#103296=CARTESIAN_POINT('Ctrl Pts',(-20.184588461652,20.7530112920262,-16.5909712942578));
#103297=CARTESIAN_POINT('Ctrl Pts',(-20.1975001920023,20.7407623758299,
-16.5899244623274));
#103298=CARTESIAN_POINT('Ctrl Pts',(-20.227213982116,20.7118533467546,-16.5875016062618));
#103299=CARTESIAN_POINT('Ctrl Pts',(-20.24389441538,20.6950713198551,-16.586130917355));
#103300=CARTESIAN_POINT('Ctrl Pts',(-20.3005974538237,20.6360770734237,
-16.5814288147065));
#103301=CARTESIAN_POINT('Ctrl Pts',(-20.339160850276,20.5924961570511,-16.5781560024563));
#103302=CARTESIAN_POINT('Ctrl Pts',(-20.4801364601401,20.4192928289693,
-16.5657682510421));
#103303=CARTESIAN_POINT('Ctrl Pts',(-20.569035385705,20.2794581754388,-16.5570654750764));
#103304=CARTESIAN_POINT('Ctrl Pts',(-20.6663071211393,20.0777938445973,
-16.5445283610871));
#103305=CARTESIAN_POINT('Ctrl Pts',(-20.6896202179217,20.0238287764598,
-16.5411692222945));
#103306=CARTESIAN_POINT('Ctrl Pts',(-20.7138514252563,19.9606378849833,
-16.5371546651799));
#103307=CARTESIAN_POINT('Ctrl Pts',(-20.7169935338606,19.9522862220692,
-16.536622475451));
#103308=CARTESIAN_POINT('Ctrl Pts',(-20.721649858507,19.939668327278,-16.5358156634409));
#103309=CARTESIAN_POINT('Ctrl Pts',(-20.7232033880908,19.9354165729295,
-16.5355433269061));
#103310=CARTESIAN_POINT('Ctrl Pts',(-20.7259567193341,19.9278055194853,
-16.5350549211475));
#103311=CARTESIAN_POINT('Ctrl Pts',(-20.7271616776866,19.9244481416342,
-16.5348391626884));
#103312=CARTESIAN_POINT('Ctrl Pts',(-20.7297493394559,19.9171804133919,
-16.5343714183857));
#103313=CARTESIAN_POINT('Ctrl Pts',(-20.7311290194295,19.9132690946268,
-16.5341192631044));
#103314=CARTESIAN_POINT('Ctrl Pts',(-20.7349423505326,19.9023563858777,
-16.5334146049514));
#103315=CARTESIAN_POINT('Ctrl Pts',(-20.7373507096332,19.8953463106673,
-16.5329606475306));
#103316=CARTESIAN_POINT('Ctrl Pts',(-20.7509691776094,19.8550186845975,
-16.5303422500017));
#103317=CARTESIAN_POINT('Ctrl Pts',(-20.7613841536692,19.8214407331623,
-16.5281353059032));
#103318=CARTESIAN_POINT('Ctrl Pts',(-20.7919130222082,19.7135952627408,
-16.5209960174452));
#103319=CARTESIAN_POINT('Ctrl Pts',(-20.8088160422474,19.6384865911504,
-16.5159496203879));
#103320=CARTESIAN_POINT('Ctrl Pts',(-20.8410710378816,19.4469921103544,
-16.5031356999716));
#103321=CARTESIAN_POINT('Ctrl Pts',(-20.8509078633986,19.3299290089427,
-16.4953606780472));
#103322=CARTESIAN_POINT('Ctrl Pts',(-20.8509993557841,19.2126515476976,
-16.4878149913274));
#103323=CARTESIAN_POINT('Ctrl Pts',(-20.8509993578195,19.2126489366114,
-16.487814823329));
#103324=CARTESIAN_POINT('Ctrl Pts',(-20.8510649772153,19.1284029942412,
-16.4823944024007));
#103325=CARTESIAN_POINT('Ctrl Pts',(-20.8461018020696,19.0442181851613,
-16.4770995077269));
#103326=CARTESIAN_POINT('Ctrl Pts',(-20.8349011956226,18.9502100090101,
-16.4713271189853));
#103327=CARTESIAN_POINT('Ctrl Pts',(-20.833594095754,18.9398876758388,-16.4706951411389));
#103328=CARTESIAN_POINT('Ctrl Pts',(-20.8312616517224,18.9224977355724,
-16.4696334764133));
#103329=CARTESIAN_POINT('Ctrl Pts',(-20.8302765596053,18.9154250011086,
-16.4692025271686));
#103330=CARTESIAN_POINT('Ctrl Pts',(-20.8283990632567,18.9024267191727,
-16.4684120439715));
#103331=CARTESIAN_POINT('Ctrl Pts',(-20.8275172537553,18.8964997373783,
-16.4680521786698));
#103332=CARTESIAN_POINT('Ctrl Pts',(-20.8256463309034,18.884281180415,-16.4673114810221));
#103333=CARTESIAN_POINT('Ctrl Pts',(-20.8246539665023,18.8779901587472,
-16.4669307557886));
#103334=CARTESIAN_POINT('Ctrl Pts',(-20.8223696978179,18.8639219737229,
-16.4660807594744));
#103335=CARTESIAN_POINT('Ctrl Pts',(-20.8210627053305,18.8561473296156,
-16.4656119724461));
#103336=CARTESIAN_POINT('Ctrl Pts',(-20.8176411999454,18.8364675613506,
-16.4644276657821));
#103337=CARTESIAN_POINT('Ctrl Pts',(-20.8154680492599,18.8245728183502,
-16.4637140127177));
#103338=CARTESIAN_POINT('Ctrl Pts',(-20.8024833903227,18.7567911956213,
-16.4596587181026));
#103339=CARTESIAN_POINT('Ctrl Pts',(-20.7895226775756,18.7013368482678,
-16.4563862764759));
#103340=CARTESIAN_POINT('Ctrl Pts',(-20.7635221427499,18.6073651777507,
-16.4508784635452));
#103341=CARTESIAN_POINT('Ctrl Pts',(-20.7515806204613,18.5685797404864,
-16.4486162141156));
#103342=CARTESIAN_POINT('Ctrl Pts',(-20.7333842942261,18.5150060471336,
-16.4454901482646));
#103343=CARTESIAN_POINT('Ctrl Pts',(-20.728066946463,18.4999150047001,-16.4446094023785));
#103344=CARTESIAN_POINT('Ctrl Pts',(-20.7225806308032,18.4848897640204,
-16.4437314734851));
#103345=CARTESIAN_POINT('Origin',(-18.734,19.211,0.));
#103346=CARTESIAN_POINT('',(-20.7225806137986,18.4848897174502,-15.646496294977));
#103347=CARTESIAN_POINT('',(-20.722580613579,18.4848897168489,-15.866216451952));
#103348=CARTESIAN_POINT('',(-20.7225806137986,18.4848897174502,0.));
#103349=CARTESIAN_POINT('Ctrl Pts',(-20.722580613579,18.4848897168488,-15.866216451952));
#103350=CARTESIAN_POINT('Ctrl Pts',(-20.7307297100332,18.5072074495721,
-15.8675066849164));
#103351=CARTESIAN_POINT('Ctrl Pts',(-20.7385063121739,18.5296711603929,
-15.868797221955));
#103352=CARTESIAN_POINT('Ctrl Pts',(-20.7729860000107,18.6349799787421,
-15.8748264466111));
#103353=CARTESIAN_POINT('Ctrl Pts',(-20.794937948196,18.7192730939136,-15.8795907956239));
#103354=CARTESIAN_POINT('Ctrl Pts',(-20.8189001290662,18.8417961064723,
-15.8867186669764));
#103355=CARTESIAN_POINT('Ctrl Pts',(-20.8251640448533,18.8791075455718,
-15.8889160607276));
#103356=CARTESIAN_POINT('Ctrl Pts',(-20.8314778226034,18.9240625158185,
-15.8916170096321));
#103357=CARTESIAN_POINT('Ctrl Pts',(-20.8324907017386,18.931566453459,-15.8920696325401));
#103358=CARTESIAN_POINT('Ctrl Pts',(-20.834000499107,18.9432232351928,-15.8927757277816));
#103359=CARTESIAN_POINT('Ctrl Pts',(-20.8345254154019,18.9473724775823,
-15.8930276485012));
#103360=CARTESIAN_POINT('Ctrl Pts',(-20.8354748337427,18.9550601170607,
-15.8934955314825));
#103361=CARTESIAN_POINT('Ctrl Pts',(-20.8359026977821,18.9585980408009,
-15.8937113018391));
#103362=CARTESIAN_POINT('Ctrl Pts',(-20.8368482734237,18.9665859874486,
-15.8941994721526));
#103363=CARTESIAN_POINT('Ctrl Pts',(-20.837360790736,18.9710365575475,-15.8944721591287));
#103364=CARTESIAN_POINT('Ctrl Pts',(-20.8388276186419,18.9841399585073,
-15.8952769913044));
#103365=CARTESIAN_POINT('Ctrl Pts',(-20.8397426747612,18.9927969653412,
-15.8958112646172));
#103366=CARTESIAN_POINT('Ctrl Pts',(-20.8458591845623,19.0542888830302,
-15.8996231613316));
#103367=CARTESIAN_POINT('Ctrl Pts',(-20.8491244445647,19.1072929582799,
-15.9029969361203));
#103368=CARTESIAN_POINT('Ctrl Pts',(-20.8507874983447,19.1767948294316,
-15.90748929889));
#103369=CARTESIAN_POINT('Ctrl Pts',(-20.8509892979912,19.1932348606781,
-15.9085569697079));
#103370=CARTESIAN_POINT('Ctrl Pts',(-20.8510113338606,19.2284498580906,
-15.910852706117));
#103371=CARTESIAN_POINT('Ctrl Pts',(-20.8507733280713,19.2472234825081,
-15.9120819250805));
#103372=CARTESIAN_POINT('Ctrl Pts',(-20.8462294560163,19.4220903742844,
-15.9235687404762));
#103373=CARTESIAN_POINT('Ctrl Pts',(-20.8249133703867,19.5772840818688,
-15.9339904580781));
#103374=CARTESIAN_POINT('Ctrl Pts',(-20.7855430759336,19.7333821023551,
-15.9442509355322));
#103375=CARTESIAN_POINT('Ctrl Pts',(-20.784353024173,19.7380337086545,-15.9445565309553));
#103376=CARTESIAN_POINT('Ctrl Pts',(-20.7672421603605,19.8039805098056,
-15.9488867117748));
#103377=CARTESIAN_POINT('Ctrl Pts',(-20.7485934598733,19.864539659252,-15.9528332812358));
#103378=CARTESIAN_POINT('Ctrl Pts',(-20.7230405459961,19.9359574164032,
-15.9574537212672));
#103379=CARTESIAN_POINT('Ctrl Pts',(-20.718721079733,19.9477006145155,-15.9582123980706));
#103380=CARTESIAN_POINT('Ctrl Pts',(-20.7114648628223,19.9669007387437,
-15.9594512520348));
#103381=CARTESIAN_POINT('Ctrl Pts',(-20.7085894774242,19.9743803828571,
-15.9599334664468));
#103382=CARTESIAN_POINT('Ctrl Pts',(-20.7033486448,19.9877854382339,-15.9607970376303));
#103383=CARTESIAN_POINT('Ctrl Pts',(-20.7009987608544,19.9937167929752,
-15.9611789113749));
#103384=CARTESIAN_POINT('Ctrl Pts',(-20.6959424920753,20.0063127670094,
-15.9619894127401));
#103385=CARTESIAN_POINT('Ctrl Pts',(-20.6932288753261,20.0129744108306,
-15.9624177907137));
#103386=CARTESIAN_POINT('Ctrl Pts',(-20.6858435314514,20.0308434331864,
-15.9635662045171));
#103387=CARTESIAN_POINT('Ctrl Pts',(-20.6811092070372,20.0420247717955,
-15.9642841130527));
#103388=CARTESIAN_POINT('Ctrl Pts',(-20.6571530390825,20.0972747076518,
-15.9678287989931));
#103389=CARTESIAN_POINT('Ctrl Pts',(-20.6365292042092,20.140722332489,-15.9706072964359));
#103390=CARTESIAN_POINT('Ctrl Pts',(-20.537430530737,20.3323544925586,-15.9828819631902));
#103391=CARTESIAN_POINT('Ctrl Pts',(-20.4430046554724,20.4715959672653,
-15.9918001711245));
#103392=CARTESIAN_POINT('Ctrl Pts',(-20.2684506691017,20.6728123011067,
-16.006384006276));
#103393=CARTESIAN_POINT('Ctrl Pts',(-20.1986341131656,20.7427558065264,
-16.0118767442219));
#103394=CARTESIAN_POINT('Ctrl Pts',(-20.1168931570434,20.8139315365527,
-16.0182979854958));
#103395=CARTESIAN_POINT('Ctrl Pts',(-20.1095379821638,20.8202477268045,
-16.0188757238266));
#103396=CARTESIAN_POINT('Ctrl Pts',(-20.0986146029711,20.829498478691,-16.0197341066941));
#103397=CARTESIAN_POINT('Ctrl Pts',(-20.0950796402505,20.832472340848,-16.0200119478965));
#103398=CARTESIAN_POINT('Ctrl Pts',(-20.0887912537901,20.8377275261928,
-16.02050636037));
#103399=CARTESIAN_POINT('Ctrl Pts',(-20.0860417540102,20.840013468644,-16.0207225896597));
#103400=CARTESIAN_POINT('Ctrl Pts',(-20.0801385590999,20.8448961619581,
-16.0211869705248));
#103401=CARTESIAN_POINT('Ctrl Pts',(-20.0769831828514,20.8474907143895,
-16.0214352683525));
#103402=CARTESIAN_POINT('Ctrl Pts',(-20.0683014447642,20.8545873765871,
-16.0221186008423));
#103403=CARTESIAN_POINT('Ctrl Pts',(-20.0627598822913,20.8590706847272,
-16.0225549530334));
#103404=CARTESIAN_POINT('Ctrl Pts',(-20.0330577939349,20.8828534781246,
-16.0248942170763));
#103405=CARTESIAN_POINT('Ctrl Pts',(-20.0085005716585,20.901648770122,-16.0268299014795));
#103406=CARTESIAN_POINT('Ctrl Pts',(-19.932933751769,20.9569030366703,-16.0327692717061));
#103407=CARTESIAN_POINT('Ctrl Pts',(-19.8807099081991,20.9916388860111,
-16.0368503877224));
#103408=CARTESIAN_POINT('Ctrl Pts',(-19.7118261425579,21.0934557365582,
-16.0498094075512));
#103409=CARTESIAN_POINT('Ctrl Pts',(-19.5902575871588,21.1517760577781,
-16.0587750607433));
#103410=CARTESIAN_POINT('Ctrl Pts',(-19.4256423433035,21.2122464581395,
-16.070068511563));
#103411=CARTESIAN_POINT('Ctrl Pts',(-19.3869104230107,21.2252156826393,
-16.0726704582485));
#103412=CARTESIAN_POINT('Ctrl Pts',(-19.3014161601891,21.2511175062419,
-16.0782894329313));
#103413=CARTESIAN_POINT('Ctrl Pts',(-19.2545345849612,21.263580056514,-16.0812910430167));
#103414=CARTESIAN_POINT('Ctrl Pts',(-19.1949880136887,21.2772375603902,
-16.0850069101745));
#103415=CARTESIAN_POINT('Ctrl Pts',(-19.182687825865,21.279943414016,-16.0857693783274));
#103416=CARTESIAN_POINT('Ctrl Pts',(-19.1631556912682,21.2840578038541,
-16.0869722487119));
#103417=CARTESIAN_POINT('Ctrl Pts',(-19.1559394242275,21.2855385968664,
-16.0874149563323));
#103418=CARTESIAN_POINT('Ctrl Pts',(-19.1424772963141,21.2882279043537,
-16.0882377213378));
#103419=CARTESIAN_POINT('Ctrl Pts',(-19.1362334522104,21.2894459866734,
-16.0886180804136));
#103420=CARTESIAN_POINT('Ctrl Pts',(-19.1223512244561,21.2920893062284,
-16.0894610260287));
#103421=CARTESIAN_POINT('Ctrl Pts',(-19.1147102694432,21.2935006764078,
-16.0899231659309));
#103422=CARTESIAN_POINT('Ctrl Pts',(-19.0924792090676,21.2974805580513,
-16.0912625446952));
#103423=CARTESIAN_POINT('Ctrl Pts',(-19.0778695114745,21.2999380647179,
-16.0921362521435));
#103424=CARTESIAN_POINT('Ctrl Pts',(-18.9612382451843,21.3182999217235,
-16.099061874341));
#103425=CARTESIAN_POINT('Ctrl Pts',(-18.8581967684149,21.3268755546564,
-16.1048707616966));
#103426=CARTESIAN_POINT('Ctrl Pts',(-18.5952918642965,21.3294748462361,
-16.1193460729866));
#103427=CARTESIAN_POINT('Ctrl Pts',(-18.43600367459,21.3129909410084,-16.1277744129058));
#103428=CARTESIAN_POINT('Ctrl Pts',(-18.2326864338793,21.268359863854,-16.1395294966699));
#103429=CARTESIAN_POINT('Ctrl Pts',(-18.1856534243482,21.2563264154215,
-16.1423242868963));
#103430=CARTESIAN_POINT('Ctrl Pts',(-18.1316337975706,21.240508352135,-16.1456660238248));
#103431=CARTESIAN_POINT('Ctrl Pts',(-18.1242001908566,21.2382871976641,
-16.1461288129868));
#103432=CARTESIAN_POINT('Ctrl Pts',(-18.1123333597317,21.2346702273449,
-16.1468725470988));
#103433=CARTESIAN_POINT('Ctrl Pts',(-18.1078921519508,21.2333005618189,
-16.147152004985));
#103434=CARTESIAN_POINT('Ctrl Pts',(-18.1000300681276,21.2308475193983,
-16.1476487500638));
#103435=CARTESIAN_POINT('Ctrl Pts',(-18.0966073939111,21.2297700566625,
-16.1478656887423));
#103436=CARTESIAN_POINT('Ctrl Pts',(-18.0893538583262,21.227466347509,-16.1483269153705));
#103437=CARTESIAN_POINT('Ctrl Pts',(-18.0855238073938,21.2262379029809,
-16.1485713256125));
#103438=CARTESIAN_POINT('Ctrl Pts',(-18.075186052926,21.222889665751,-16.1492333274271));
#103439=CARTESIAN_POINT('Ctrl Pts',(-18.0686851558668,21.2207492378983,
-16.1496521053904));
#103440=CARTESIAN_POINT('Ctrl Pts',(-18.036345475416,21.2099272570659,-16.1517473413617));
#103441=CARTESIAN_POINT('Ctrl Pts',(-18.0106669607787,21.2007791751567,
-16.1534491360682));
#103442=CARTESIAN_POINT('Ctrl Pts',(-17.9367523830499,21.1728269973373,
-16.1584445029613));
#103443=CARTESIAN_POINT('Ctrl Pts',(-17.8890221570268,21.1527468047928,
-16.161791281838));
#103444=CARTESIAN_POINT('Ctrl Pts',(-17.7166761289524,21.0726822901161,
-16.1742133112566));
#103445=CARTESIAN_POINT('Ctrl Pts',(-17.5972714955827,21.0022736173384,
-16.1834597839596));
#103446=CARTESIAN_POINT('Ctrl Pts',(-17.4529915619666,20.8969226903731,
-16.1950273585044));
#103447=CARTESIAN_POINT('Ctrl Pts',(-17.4210820545858,20.8721937561901,
-16.1976159110248));
#103448=CARTESIAN_POINT('Ctrl Pts',(-17.3444281223032,20.8091998424504,
-16.2039028856977));
#103449=CARTESIAN_POINT('Ctrl Pts',(-17.3005335187298,20.7699508192764,
-16.2075631952157));
#103450=CARTESIAN_POINT('Ctrl Pts',(-17.2495685115031,20.7204043217027,
-16.2118911509734));
#103451=CARTESIAN_POINT('Ctrl Pts',(-17.240882618768,20.7118126952076,-16.2126317007576));
#103452=CARTESIAN_POINT('Ctrl Pts',(-17.2266874285987,20.6975263456261,
-16.2138470137106));
#103453=CARTESIAN_POINT('Ctrl Pts',(-17.221134949198,20.6918751145416,-16.2143236849716));
#103454=CARTESIAN_POINT('Ctrl Pts',(-17.2111742270243,20.6816227471235,
-16.2151812099355));
#103455=CARTESIAN_POINT('Ctrl Pts',(-17.2067548074559,20.6770326471202,
-16.2155625508318));
#103456=CARTESIAN_POINT('Ctrl Pts',(-17.1973490510837,20.6671749449462,
-16.21637605918));
#103457=CARTESIAN_POINT('Ctrl Pts',(-17.1923689165333,20.6619015175376,
-16.2168079553886));
#103458=CARTESIAN_POINT('Ctrl Pts',(-17.1789387457425,20.6475331919123,
-16.2179759198169));
#103459=CARTESIAN_POINT('Ctrl Pts',(-17.1705413646107,20.6383893026341,
-16.2187097318021));
#103460=CARTESIAN_POINT('Ctrl Pts',(-17.1276891071625,20.5908956837354,
-16.2224736412004));
#103461=CARTESIAN_POINT('Ctrl Pts',(-17.0945613355072,20.5513687107548,
-16.225447785162));
#103462=CARTESIAN_POINT('Ctrl Pts',(-16.9568346737977,20.3742821172794,
-16.2381786686098));
#103463=CARTESIAN_POINT('Ctrl Pts',(-16.8678615545447,20.2254304265473,
-16.247331349834));
#103464=CARTESIAN_POINT('Ctrl Pts',(-16.7616825013397,19.9854006088846,
-16.2617545809859));
#103465=CARTESIAN_POINT('Ctrl Pts',(-16.7306535929744,19.9011679363643,
-16.26677469244));
#103466=CARTESIAN_POINT('Ctrl Pts',(-16.7023069985309,19.8059837817041,
-16.2726590244218));
#103467=CARTESIAN_POINT('Ctrl Pts',(-16.6996155989034,19.7967151639812,
-16.2732342028016));
#103468=CARTESIAN_POINT('Ctrl Pts',(-16.6957321970007,19.7829918053178,
-16.2740894950867));
#103469=CARTESIAN_POINT('Ctrl Pts',(-16.6944911781576,19.778550902386,-16.2743668346848));
#103470=CARTESIAN_POINT('Ctrl Pts',(-16.6923138083745,19.7706599632556,
-16.2748606939627));
#103471=CARTESIAN_POINT('Ctrl Pts',(-16.6913716771482,19.7672115730687,
-16.2750768745022));
#103472=CARTESIAN_POINT('Ctrl Pts',(-16.6893702219578,19.7598121744544,
-16.2755415352424));
#103473=CARTESIAN_POINT('Ctrl Pts',(-16.6883136293299,19.7558605365472,
-16.2757901637037));
#103474=CARTESIAN_POINT('Ctrl Pts',(-16.6854410361121,19.7449909435058,
-16.2764753171759));
#103475=CARTESIAN_POINT('Ctrl Pts',(-16.683648651203,19.7380668832247,-16.2769131711832));
#103476=CARTESIAN_POINT('Ctrl Pts',(-16.6742110604741,19.7008323217873,
-16.2792747866716));
#103477=CARTESIAN_POINT('Ctrl Pts',(-16.6672032640702,19.6703660748689,
-16.2812320516721));
#103478=CARTESIAN_POINT('Ctrl Pts',(-16.6276983622846,19.4793522263671,
-16.2936116224414));
#103479=CARTESIAN_POINT('Ctrl Pts',(-16.6132527178837,19.3156433572303,
-16.3046448268863));
#103480=CARTESIAN_POINT('Ctrl Pts',(-16.6210948451834,19.0348061329448,
-16.3229983368271));
#103481=CARTESIAN_POINT('Ctrl Pts',(-16.6340792518069,18.9181635375945,
-16.3304615466166));
#103482=CARTESIAN_POINT('Ctrl Pts',(-16.6594067217434,18.7891516385093,
-16.3384894193511));
#103483=CARTESIAN_POINT('Ctrl Pts',(-16.6623023195749,18.7751536429743,
-16.3393576643713));
#103484=CARTESIAN_POINT('Ctrl Pts',(-16.6671361852646,18.7529230724605,
-16.3407323170003));
#103485=CARTESIAN_POINT('Ctrl Pts',(-16.6689823540701,18.7446711187955,
-16.3412416549584));
#103486=CARTESIAN_POINT('Ctrl Pts',(-16.672325390675,18.7301377565633,-16.3421371230851));
#103487=CARTESIAN_POINT('Ctrl Pts',(-16.6738016388605,18.7238517616893,
-16.3425239097957));
#103488=CARTESIAN_POINT('Ctrl Pts',(-16.67691430618,18.7108649938352,-16.3433219614256));
#103489=CARTESIAN_POINT('Ctrl Pts',(-16.6785547625418,18.7041652600187,
-16.3437330911813));
#103490=CARTESIAN_POINT('Ctrl Pts',(-16.6828492642127,18.6869900426648,
-16.3447856330288));
#103491=CARTESIAN_POINT('Ctrl Pts',(-16.6855508476377,18.6765265646941,
-16.3454255047846));
#103492=CARTESIAN_POINT('Ctrl Pts',(-16.6971573633127,18.6329545722423,
-16.3480848382461));
#103493=CARTESIAN_POINT('Ctrl Pts',(-16.7067860851717,18.6000430596461,
-16.350080801271));
#103494=CARTESIAN_POINT('Ctrl Pts',(-16.7339499873085,18.514924902796,-16.3552212001254));
#103495=CARTESIAN_POINT('Ctrl Pts',(-16.7527303146239,18.4631419438977,
-16.3583263208017));
#103496=CARTESIAN_POINT('Ctrl Pts',(-16.8147573454043,18.3109194007014,
-16.3674664772092));
#103497=CARTESIAN_POINT('Ctrl Pts',(-16.8637846761917,18.2130355803018,
-16.3733527694772));
#103498=CARTESIAN_POINT('Ctrl Pts',(-16.9417130856346,18.0835493053502,
-16.381580605132));
#103499=CARTESIAN_POINT('Ctrl Pts',(-16.9643308080253,18.0483701229774,
-16.3838660861657));
#103500=CARTESIAN_POINT('Ctrl Pts',(-17.0313688610994,17.9505932973252,
-16.3904244396197));
#103501=CARTESIAN_POINT('Ctrl Pts',(-17.0781674680437,17.8897150961318,
-16.3947571235019));
#103502=CARTESIAN_POINT('Ctrl Pts',(-17.1343529255045,17.8243102223344,
-16.3998672466576));
#103503=CARTESIAN_POINT('Ctrl Pts',(-17.140593455917,17.8171438811401,-16.4004336703677));
#103504=CARTESIAN_POINT('Ctrl Pts',(-17.1499141495439,17.8065848145464,
-16.4012783851386));
#103505=CARTESIAN_POINT('Ctrl Pts',(-17.1529575211923,17.803159570815,-16.4015540000756));
#103506=CARTESIAN_POINT('Ctrl Pts',(-17.1583931390188,17.797081763818,-16.4020459658933));
#103507=CARTESIAN_POINT('Ctrl Pts',(-17.160781002238,17.7944253483032,-16.4022619874058));
#103508=CARTESIAN_POINT('Ctrl Pts',(-17.1659305135167,17.7887257744956,
-16.4027276495945));
#103509=CARTESIAN_POINT('Ctrl Pts',(-17.1686942620905,17.7856846548296,
-16.4029774455902));
#103510=CARTESIAN_POINT('Ctrl Pts',(-17.176350428545,17.7773092371958,-16.4036690391799));
#103511=CARTESIAN_POINT('Ctrl Pts',(-17.1812613228103,17.7719920126428,
-16.404112206673));
#103512=CARTESIAN_POINT('Ctrl Pts',(-17.2083631610853,17.7429480128418,
-16.4065549887513));
#103513=CARTESIAN_POINT('Ctrl Pts',(-17.2310694535619,17.7197106565648,
-16.4085908318708));
#103514=CARTESIAN_POINT('Ctrl Pts',(-17.370688834416,17.5832537899217,-16.4209957699345));
#103515=CARTESIAN_POINT('Ctrl Pts',(-17.4998028544643,17.4833043126514,
-16.4319555752646));
#103516=CARTESIAN_POINT('Ctrl Pts',(-17.7390722945051,17.3387140770515,
-16.4502166179063));
#103517=CARTESIAN_POINT('Ctrl Pts',(-17.8438954085251,17.2866670401905,
-16.4576579831164));
#103518=CARTESIAN_POINT('Ctrl Pts',(-17.9657768170427,17.2382540960564,
-16.4656656888531));
#103519=CARTESIAN_POINT('Ctrl Pts',(-17.979112634985,17.2331126568417,-16.4665338263646));
#103520=CARTESIAN_POINT('Ctrl Pts',(-18.0004194121345,17.2251450171892,
-16.4679083414871));
#103521=CARTESIAN_POINT('Ctrl Pts',(-18.0083568249097,17.2222309140243,
-16.4684176485354));
#103522=CARTESIAN_POINT('Ctrl Pts',(-18.0223860568188,17.21717546241,-16.4693130807066));
#103523=CARTESIAN_POINT('Ctrl Pts',(-18.0284705731536,17.2150142986202,
-16.4696998622056));
#103524=CARTESIAN_POINT('Ctrl Pts',(-18.0410753379798,17.2106020416654,
-16.470497920687));
#103525=CARTESIAN_POINT('Ctrl Pts',(-18.0475968988859,17.2083549082632,
-16.4709090624189));
#103526=CARTESIAN_POINT('Ctrl Pts',(-18.0643641600255,17.2026689420415,
-16.4719616713599));
#103527=CARTESIAN_POINT('Ctrl Pts',(-18.0746255008292,17.199276591343,-16.4726015978474));
#103528=CARTESIAN_POINT('Ctrl Pts',(-18.1175537188811,17.1854484740681,
-16.4752614630592));
#103529=CARTESIAN_POINT('Ctrl Pts',(-18.1504468343376,17.1757282980023,
-16.4772578911056));
#103530=CARTESIAN_POINT('Ctrl Pts',(-18.2367466174557,17.1524904298777,
-16.4823997581472));
#103531=CARTESIAN_POINT('Ctrl Pts',(-18.2904712283545,17.1402500271525,
-16.4855058525303));
#103532=CARTESIAN_POINT('Ctrl Pts',(-18.4520739380687,17.11001013454,-16.4946477078393));
#103533=CARTESIAN_POINT('Ctrl Pts',(-18.5609318159898,17.0982555741269,
-16.5005347309068));
#103534=CARTESIAN_POINT('Ctrl Pts',(-18.7136383447923,17.0936521009622,
-16.5088523812844));
#103535=CARTESIAN_POINT('Ctrl Pts',(-18.7570954580702,17.0936802025071,
-16.5112275099705));
#103536=CARTESIAN_POINT('Ctrl Pts',(-18.8293122726157,17.0959504959802,
-16.5152284126781));
#103537=CARTESIAN_POINT('Ctrl Pts',(-18.8580825128274,17.0974432210305,
-16.51683663935));
#103538=CARTESIAN_POINT('Ctrl Pts',(-18.9344037809975,17.1029667625486,
-16.5211610610238));
#103539=CARTESIAN_POINT('Ctrl Pts',(-18.9818612852048,17.1080188216196,
-16.5239101472252));
#103540=CARTESIAN_POINT('Ctrl Pts',(-19.0367559107812,17.1157464166713,
-16.527201522163));
#103541=CARTESIAN_POINT('Ctrl Pts',(-19.0444022413434,17.1168655333508,
-16.5276625120003));
#103542=CARTESIAN_POINT('Ctrl Pts',(-19.0566281874649,17.1187233523931,
-16.5284039007429));
#103543=CARTESIAN_POINT('Ctrl Pts',(-19.0612118812146,17.1194352983179,
-16.5286828273594));
#103544=CARTESIAN_POINT('Ctrl Pts',(-19.0693359648415,17.1207245018154,
-16.5291789709452));
#103545=CARTESIAN_POINT('Ctrl Pts',(-19.0728772703606,17.1212956996041,
-16.5293958423454));
#103546=CARTESIAN_POINT('Ctrl Pts',(-19.0803914668496,17.1225273113743,
-16.5298573134428));
#103547=CARTESIAN_POINT('Ctrl Pts',(-19.0843638679602,17.1231900520296,
-16.5301020373918));
#103548=CARTESIAN_POINT('Ctrl Pts',(-19.0951045385767,17.1250135021463,
-16.5307657556233));
#103549=CARTESIAN_POINT('Ctrl Pts',(-19.1018690225466,17.126195803853,-16.5311859466335));
#103550=CARTESIAN_POINT('Ctrl Pts',(-19.1357278993662,17.1322836009826,
-16.5332996893001));
#103551=CARTESIAN_POINT('Ctrl Pts',(-19.1627291616918,17.1376842231241,
-16.5350191066817));
#103552=CARTESIAN_POINT('Ctrl Pts',(-19.2409367409709,17.1549197745823,
-16.5400829862256));
#103553=CARTESIAN_POINT('Ctrl Pts',(-19.2918153599703,17.168136316274,-16.5434822691979));
#103554=CARTESIAN_POINT('Ctrl Pts',(-19.4882268235893,17.2270418490906,
-16.5568920889005));
#103555=CARTESIAN_POINT('Ctrl Pts',(-19.6291636099585,17.2865162912103,
-16.5671007364737));
#103556=CARTESIAN_POINT('Ctrl Pts',(-19.8338772340138,17.4003011684494,
-16.582152932376));
#103557=CARTESIAN_POINT('Ctrl Pts',(-19.9029181156154,17.4440836420308,
-16.5872827356465));
#103558=CARTESIAN_POINT('Ctrl Pts',(-19.980145983803,17.4995711363689,-16.5930824131077));
#103559=CARTESIAN_POINT('Ctrl Pts',(-19.9909542816557,17.5074934649361,
-16.5938956881502));
#103560=CARTESIAN_POINT('Ctrl Pts',(-20.0082492474889,17.5204246554479,
-16.59519982845));
#103561=CARTESIAN_POINT('Ctrl Pts',(-20.0147831966166,17.5253693920239,
-16.5956931745885));
#103562=CARTESIAN_POINT('Ctrl Pts',(-20.0262334353305,17.5341396751493,
-16.5965589317974));
#103563=CARTESIAN_POINT('Ctrl Pts',(-20.0311618251205,17.5379491934851,
-16.5969319672758));
#103564=CARTESIAN_POINT('Ctrl Pts',(-20.0413907327298,17.5459282446111,
-16.5977070716508));
#103565=CARTESIAN_POINT('Ctrl Pts',(-20.0466882917616,17.5501014694114,
-16.5981089881652));
#103566=CARTESIAN_POINT('Ctrl Pts',(-20.0602606723611,17.5608987978843,
-16.5991400248028));
#103567=CARTESIAN_POINT('Ctrl Pts',(-20.0685059138941,17.5675599127918,
-16.5997676569238));
#103568=CARTESIAN_POINT('Ctrl Pts',(-20.0863401697637,17.5821904615574,
-16.6011282274808));
#103569=CARTESIAN_POINT('Ctrl Pts',(-20.0959095466504,17.5901832787685,
-16.6018602022666));
#103570=CARTESIAN_POINT('Ctrl Pts',(-20.1234422522698,17.6135959659674,
-16.6039724090936));
#103571=CARTESIAN_POINT('Ctrl Pts',(-20.1412185737194,17.6292334655892,
-16.6053438806744));
#103572=CARTESIAN_POINT('Ctrl Pts',(-20.2017877841306,17.6843445119854,
-16.6100495124582));
#103573=CARTESIAN_POINT('Ctrl Pts',(-20.243213840497,17.7252839156753,-16.6133249691915));
#103574=CARTESIAN_POINT('Ctrl Pts',(-20.3957047322489,17.8889526915444,
-16.6257330304248));
#103575=CARTESIAN_POINT('Ctrl Pts',(-20.49391370683,18.0228211486623,-16.6344517680048));
#103576=CARTESIAN_POINT('Ctrl Pts',(-20.604329376699,18.2175383461647,-16.6469895627226));
#103577=CARTESIAN_POINT('Ctrl Pts',(-20.631013692211,18.2694928112654,-16.6503279516777));
#103578=CARTESIAN_POINT('Ctrl Pts',(-20.6592540855346,18.3305653946573,
-16.6543193806578));
#103579=CARTESIAN_POINT('Ctrl Pts',(-20.6629425174268,18.3386760084038,
-16.6548507894081));
#103580=CARTESIAN_POINT('Ctrl Pts',(-20.668426287038,18.3509393011937,-16.6556566447636));
#103581=CARTESIAN_POINT('Ctrl Pts',(-20.670259744806,18.3550749650901,-16.6559288136484));
#103582=CARTESIAN_POINT('Ctrl Pts',(-20.6735150751846,18.3624818823369,
-16.6564170388211));
#103583=CARTESIAN_POINT('Ctrl Pts',(-20.6749419487363,18.3657508803674,
-16.6566327852967));
#103584=CARTESIAN_POINT('Ctrl Pts',(-20.6780109534993,18.3728307857159,
-16.6571006427445));
#103585=CARTESIAN_POINT('Ctrl Pts',(-20.679650120897,18.3766428669508,-16.6573529239024));
#103586=CARTESIAN_POINT('Ctrl Pts',(-20.6841897084988,18.3872863472987,
-16.658058281148));
#103587=CARTESIAN_POINT('Ctrl Pts',(-20.6870653953247,18.3941281381909,
-16.6585128163782));
#103588=CARTESIAN_POINT('Ctrl Pts',(-20.7013913801506,18.4287204088161,
-16.6608160793144));
#103589=CARTESIAN_POINT('Ctrl Pts',(-20.7122856338737,18.4566951057172,
-16.6626952662248));
#103590=CARTESIAN_POINT('Ctrl Pts',(-20.7225806137285,18.4848897172584,
-16.6645990097762));
#103591=CARTESIAN_POINT('Ctrl Pts',(-20.7225806308032,18.4848897640204,
-16.4437314734851));
#103592=CARTESIAN_POINT('Ctrl Pts',(-20.6771293833756,18.3604135263889,
-16.436458293116));
#103593=CARTESIAN_POINT('Ctrl Pts',(-20.6200812694952,18.2404523288822,
-16.4293983522549));
#103594=CARTESIAN_POINT('Ctrl Pts',(-20.5206824853801,18.0737957523732,
-16.4185943630028));
#103595=CARTESIAN_POINT('Ctrl Pts',(-20.4869124077141,18.0224023035683,
-16.4151049135036));
#103596=CARTESIAN_POINT('Ctrl Pts',(-20.4434978721318,17.9622131288376,
-16.4107316457269));
#103597=CARTESIAN_POINT('Ctrl Pts',(-20.4359446106736,17.9519383856621,
-16.4099745467869));
#103598=CARTESIAN_POINT('Ctrl Pts',(-20.4252035008078,17.9376004639855,
-16.4089021658407));
#103599=CARTESIAN_POINT('Ctrl Pts',(-20.4220927372145,17.9334795231593,
-16.4085920806201));
#103600=CARTESIAN_POINT('Ctrl Pts',(-20.4167518697292,17.9264578510226,
-16.4080604506043));
#103601=CARTESIAN_POINT('Ctrl Pts',(-20.4145292380405,17.9235514117181,
-16.407839430319));
#103602=CARTESIAN_POINT('Ctrl Pts',(-20.4102412287356,17.9179741913383,
-16.4074134205317));
#103603=CARTESIAN_POINT('Ctrl Pts',(-20.4081769867017,17.9153025755965,
-16.4072085158136));
#103604=CARTESIAN_POINT('Ctrl Pts',(-20.4026652060468,17.9082041940133,
-16.4066618876494));
#103605=CARTESIAN_POINT('Ctrl Pts',(-20.3992064723666,17.9037862130834,
-16.4063193790731));
#103606=CARTESIAN_POINT('Ctrl Pts',(-20.3867300072992,17.8879793843973,
-16.4050858505679));
#103607=CARTESIAN_POINT('Ctrl Pts',(-20.3776129039418,17.8766699727079,
-16.4041881384434));
#103608=CARTESIAN_POINT('Ctrl Pts',(-20.2674959835265,17.7429152295266,
-16.3933979815739));
#103609=CARTESIAN_POINT('Ctrl Pts',(-20.1531580344548,17.6321183781371,
-16.3827537690552));
#103610=CARTESIAN_POINT('Ctrl Pts',(-19.950393656403,17.47561281834,-16.3658987455293));
#103611=CARTESIAN_POINT('Ctrl Pts',(-19.8692390903128,17.4214698469529,
-16.359573034508));
#103612=CARTESIAN_POINT('Ctrl Pts',(-19.7557131161288,17.3565725621692,
-16.3513405752646));
#103613=CARTESIAN_POINT('Ctrl Pts',(-19.7264039572586,17.3407237121442,
-16.3492658339167));
#103614=CARTESIAN_POINT('Ctrl Pts',(-19.6825420963165,17.3183270938211,
-16.3462343591232));
#103615=CARTESIAN_POINT('Ctrl Pts',(-19.668270949049,17.3112419486188,-16.3452592206358));
#103616=CARTESIAN_POINT('Ctrl Pts',(-19.6422520423826,17.2986885492985,
-16.3435012913826));
#103617=CARTESIAN_POINT('Ctrl Pts',(-19.6305315871073,17.2931658095658,
-16.3427166413518));
#103618=CARTESIAN_POINT('Ctrl Pts',(-19.6120993731491,17.2846863549306,
-16.3414937453226));
#103619=CARTESIAN_POINT('Ctrl Pts',(-19.605421842518,17.2816563958703,-16.3410529780408));
#103620=CARTESIAN_POINT('Ctrl Pts',(-19.5986901532814,17.2786439405234,
-16.3406108755786));
#103621=CARTESIAN_POINT('Ctrl Pts',(-19.5986516685325,17.2786267198386,
-16.3406083481732));
#103622=CARTESIAN_POINT('Ctrl Pts',(-19.5985733693193,17.2785916862717,
-16.3406032061855));
#103623=CARTESIAN_POINT('Ctrl Pts',(-19.5985335547086,17.2785738734209,
-16.3406005915987));
#103624=CARTESIAN_POINT('Ctrl Pts',(-19.5984525465977,17.2785376338161,
-16.3405952720348));
#103625=CARTESIAN_POINT('Ctrl Pts',(-19.5984113529341,17.2785192070928,
-16.3405925670524));
#103626=CARTESIAN_POINT('Ctrl Pts',(-19.5983275352937,17.2784817170559,
-16.3405870633372));
#103627=CARTESIAN_POINT('Ctrl Pts',(-19.5982849113589,17.2784626538725,
-16.3405842646131));
#103628=CARTESIAN_POINT('Ctrl Pts',(-19.598198170761,17.2784238633397,-16.3405785693342));
#103629=CARTESIAN_POINT('Ctrl Pts',(-19.5981540675683,17.2784041421348,
-16.3405756736706));
#103630=CARTESIAN_POINT('Ctrl Pts',(-19.598064318164,17.2783640134328,-16.3405697812296));
#103631=CARTESIAN_POINT('Ctrl Pts',(-19.5980186708474,17.2783436055714,
-16.3405667843869));
#103632=CARTESIAN_POINT('Ctrl Pts',(-19.597925780192,17.2783020802525,-16.3405606861292));
#103633=CARTESIAN_POINT('Ctrl Pts',(-19.59787853576,17.2782809624444,-16.3405575846498));
#103634=CARTESIAN_POINT('Ctrl Pts',(-19.5977823906201,17.2782379907184,
-16.3405512731856));
#103635=CARTESIAN_POINT('Ctrl Pts',(-19.5977334888798,17.2782161364872,
-16.340548063141));
#103636=CARTESIAN_POINT('Ctrl Pts',(-19.5976339663508,17.2781716643121,
-16.3405415304496));
#103637=CARTESIAN_POINT('Ctrl Pts',(-19.5975833446291,17.2781490461103,
-16.3405382077501));
#103638=CARTESIAN_POINT('Ctrl Pts',(-19.5974803168117,17.2781030172893,
-16.3405314454869));
#103639=CARTESIAN_POINT('Ctrl Pts',(-19.5974279098204,17.2780796064409,
-16.3405280058735));
#103640=CARTESIAN_POINT('Ctrl Pts',(-19.5973212434366,17.2780319624573,
-16.3405210053453));
#103641=CARTESIAN_POINT('Ctrl Pts',(-19.5972669832314,17.2780077291429,
-16.340517444387));
#103642=CARTESIAN_POINT('Ctrl Pts',(-19.5971565396027,17.2779584091577,
-16.3405101965509));
#103643=CARTESIAN_POINT('Ctrl Pts',(-19.5971003554038,17.277933322338,-16.3405065096329));
#103644=CARTESIAN_POINT('Ctrl Pts',(-19.5969859901241,17.2778822630506,
-16.3404990050754));
#103645=CARTESIAN_POINT('Ctrl Pts',(-19.5969278082144,17.277856290425,-16.3404951873928));
#103646=CARTESIAN_POINT('Ctrl Pts',(-19.5968093706668,17.2778034258661,
-16.3404874162982));
#103647=CARTESIAN_POINT('Ctrl Pts',(-19.5967491144018,17.2777765338812,
-16.3404834628571));
#103648=CARTESIAN_POINT('Ctrl Pts',(-19.5966264481866,17.2777217956127,
-16.3404754150362));
#103649=CARTESIAN_POINT('Ctrl Pts',(-19.5965640376004,17.2776939492908,
-16.3404713206277));
#103650=CARTESIAN_POINT('Ctrl Pts',(-19.5964369795317,17.2776372659672,
-16.3404629854526));
#103651=CARTESIAN_POINT('Ctrl Pts',(-19.5963723314514,17.2776084289628,
-16.3404587446608));
#103652=CARTESIAN_POINT('Ctrl Pts',(-19.5962407116536,17.2775497263845,
-16.3404501110717));
#103653=CARTESIAN_POINT('Ctrl Pts',(-19.5961737395157,17.2775198609072,
-16.3404457182618));
#103654=CARTESIAN_POINT('Ctrl Pts',(-19.5960373796211,17.277459061228,-16.3404367746491));
#103655=CARTESIAN_POINT('Ctrl Pts',(-19.59596799408,17.27742812832,-16.3404322240079));
#103656=CARTESIAN_POINT('Ctrl Pts',(-19.5958399344728,17.2773710460707,
-16.340423825675));
#103657=CARTESIAN_POINT('Ctrl Pts',(-19.5957812596592,17.2773448951206,
-16.3404199778665));
#103658=CARTESIAN_POINT('Ctrl Pts',(-19.5956540361996,17.277288199464,-16.3404116351068));
#103659=CARTESIAN_POINT('Ctrl Pts',(-19.5955854859827,17.277257655225,-16.3404071401146));
#103660=CARTESIAN_POINT('Ctrl Pts',(-19.5954368396001,17.2771914316386,
-16.3403973935395));
#103661=CARTESIAN_POINT('Ctrl Pts',(-19.5953567419957,17.2771557532451,
-16.340392141947));
#103662=CARTESIAN_POINT('Ctrl Pts',(-19.5951830437577,17.2770783946493,
-16.3403807541239));
#103663=CARTESIAN_POINT('Ctrl Pts',(-19.5950894416536,17.2770367159713,
-16.3403746179126));
#103664=CARTESIAN_POINT('Ctrl Pts',(-19.5948864441817,17.2769463439288,
-16.3403613110791));
#103665=CARTESIAN_POINT('Ctrl Pts',(-19.594777047193,17.2768976528207,-16.3403541405089));
#103666=CARTESIAN_POINT('Ctrl Pts',(-19.5945397803289,17.2767920726926,
-16.3403385898189));
#103667=CARTESIAN_POINT('Ctrl Pts',(-19.5944119093255,17.276735187241,-16.3403302098415));
#103668=CARTESIAN_POINT('Ctrl Pts',(-19.5941384637297,17.276613573095,-16.3403122914124));
#103669=CARTESIAN_POINT('Ctrl Pts',(-19.5939928874732,17.2765488481542,
-16.3403027530904));
#103670=CARTESIAN_POINT('Ctrl Pts',(-19.5879466551029,17.2738614384986,
-16.3399066404347));
#103671=CARTESIAN_POINT('Ctrl Pts',(-19.5820339878978,17.2712657261848,
-16.3395209938398));
#103672=CARTESIAN_POINT('Ctrl Pts',(-19.5683496169495,17.2653326976684,
-16.3386323563755));
#103673=CARTESIAN_POINT('Ctrl Pts',(-19.5605695715526,17.2620148073379,
-16.3381300326161));
#103674=CARTESIAN_POINT('Ctrl Pts',(-19.5395818879779,17.2532126435049,
-16.3367825932059));
#103675=CARTESIAN_POINT('Ctrl Pts',(-19.5263380737549,17.2478153669833,
-16.3359404247015));
#103676=CARTESIAN_POINT('Ctrl Pts',(-19.4044111537354,17.1995610985438,
-16.3282585996343));
#103677=CARTESIAN_POINT('Ctrl Pts',(-19.2924031978274,17.16563238037,-16.3217355538195));
#103678=CARTESIAN_POINT('Ctrl Pts',(-19.0189625714433,17.1069576579037,
-16.3064254854089));
#103679=CARTESIAN_POINT('Ctrl Pts',(-18.8563815570725,17.0912809823326,
-16.2978217993399));
#103680=CARTESIAN_POINT('Ctrl Pts',(-18.6612137518337,17.0950031886249,
-16.2866124962614));
#103681=CARTESIAN_POINT('Ctrl Pts',(-18.6288156799317,17.096366144434,-16.2847212281513));
#103682=CARTESIAN_POINT('Ctrl Pts',(-18.5892451537753,17.0989423863501,
-16.2823601438526));
#103683=CARTESIAN_POINT('Ctrl Pts',(-18.5820291404291,17.0994493415292,
-16.2819274963755));
#103684=CARTESIAN_POINT('Ctrl Pts',(-18.5707191812515,17.1003021880258,
-16.2812459236871));
#103685=CARTESIAN_POINT('Ctrl Pts',(-18.5666233246019,17.1006230367261,
-16.2809983814537));
#103686=CARTESIAN_POINT('Ctrl Pts',(-18.5589680781428,17.1012451359411,
-16.2805343425187));
#103687=CARTESIAN_POINT('Ctrl Pts',(-18.5554085080156,17.1015434732086,
-16.280318010716));
#103688=CARTESIAN_POINT('Ctrl Pts',(-18.547283294754,17.1022451826382,-16.2798229313329));
#103689=CARTESIAN_POINT('Ctrl Pts',(-18.5427182116542,17.1026543726659,
-16.2795438612244));
#103690=CARTESIAN_POINT('Ctrl Pts',(-18.5286853279181,17.1039581576354,
-16.2786832752382));
#103691=CARTESIAN_POINT('Ctrl Pts',(-18.5192223498878,17.1049017132848,
-16.2780991138915));
#103692=CARTESIAN_POINT('Ctrl Pts',(-18.4339755954835,17.1139821752215,
-16.2728041206773));
#103693=CARTESIAN_POINT('Ctrl Pts',(-18.3586841778058,17.1261417642554,
-16.2678966319496));
#103694=CARTESIAN_POINT('Ctrl Pts',(-18.1463146241132,17.1723160567457,
-16.2536806632996));
#103695=CARTESIAN_POINT('Ctrl Pts',(-18.0117386262373,17.2160188825045,
-16.2442435460687));
#103696=CARTESIAN_POINT('Ctrl Pts',(-17.8258254012171,17.2976935426875,
-16.2311229307906));
#103697=CARTESIAN_POINT('Ctrl Pts',(-17.7702537487403,17.3250739673241,
-16.2271842608108));
#103698=CARTESIAN_POINT('Ctrl Pts',(-17.6832499524569,17.3727929968713,
-16.2210008794221));
#103699=CARTESIAN_POINT('Ctrl Pts',(-17.6510201800112,17.3915947026587,
-16.218706056465));
#103700=CARTESIAN_POINT('Ctrl Pts',(-17.6098319690349,17.4171049824945,
-16.2157658600642));
#103701=CARTESIAN_POINT('Ctrl Pts',(-17.6004077915956,17.4230453562378,
-16.2150925815631));
#103702=CARTESIAN_POINT('Ctrl Pts',(-17.5851630853068,17.4328235918107,
-16.2140024688672));
#103703=CARTESIAN_POINT('Ctrl Pts',(-17.5793139433328,17.4366162456926,
-16.2135839667249));
#103704=CARTESIAN_POINT('Ctrl Pts',(-17.5681054991215,17.4439628292598,
-16.2127814967892));
#103705=CARTESIAN_POINT('Ctrl Pts',(-17.5627434554788,17.4475124161817,
-16.212397372646));
#103706=CARTESIAN_POINT('Ctrl Pts',(-17.5505086939385,17.4556920504556,
-16.2115203352037));
#103707=CARTESIAN_POINT('Ctrl Pts',(-17.5436467939402,17.4603381488533,
-16.2110280330906));
#103708=CARTESIAN_POINT('Ctrl Pts',(-17.5255013264748,17.4727802080444,
-16.2097249746757));
#103709=CARTESIAN_POINT('Ctrl Pts',(-17.5142658178665,17.4806458087434,
-16.2089168661951));
#103710=CARTESIAN_POINT('Ctrl Pts',(-17.4292845650414,17.5413773612578,
-16.2027930763984));
#103711=CARTESIAN_POINT('Ctrl Pts',(-17.3589250296735,17.5988294597261,
-16.1976619162658));
#103712=CARTESIAN_POINT('Ctrl Pts',(-17.1896366131574,17.7562337572102,
-16.1848680665584));
#103713=CARTESIAN_POINT('Ctrl Pts',(-17.0965815619116,17.8618291740648,
-16.1774026230317));
#103714=CARTESIAN_POINT('Ctrl Pts',(-16.9829794112793,18.0199644921558,
-16.1666393735447));
#103715=CARTESIAN_POINT('Ctrl Pts',(-16.9530034134662,18.0652735806959,
-16.1635936993806));
#103716=CARTESIAN_POINT('Ctrl Pts',(-16.9101883323203,18.1357361888307,
-16.158835922541));
#103717=CARTESIAN_POINT('Ctrl Pts',(-16.8960540260014,18.1600786492588,
-16.1571885311306));
#103718=CARTESIAN_POINT('Ctrl Pts',(-16.8790567968164,18.1907438779622,
-16.1550994406237));
#103719=CARTESIAN_POINT('Ctrl Pts',(-16.875733323864,18.1968097816774,-16.1546855345475));
#103720=CARTESIAN_POINT('Ctrl Pts',(-16.8705166336183,18.2064428579688,
-16.1540270028819));
#103721=CARTESIAN_POINT('Ctrl Pts',(-16.8686037616162,18.2099994097988,
-16.1537836097099));
#103722=CARTESIAN_POINT('Ctrl Pts',(-16.8650121395518,18.216723264081,-16.1533229267435));
#103723=CARTESIAN_POINT('Ctrl Pts',(-16.86333125366,18.2198893649859,-16.1531057752928));
#103724=CARTESIAN_POINT('Ctrl Pts',(-16.8595026039966,18.2271454106509,
-16.1526076040898));
#103725=CARTESIAN_POINT('Ctrl Pts',(-16.8573601830321,18.2312381222744,
-16.1523262515481));
#103726=CARTESIAN_POINT('Ctrl Pts',(-16.8516996201043,18.2421382972362,
-16.1515760239232));
#103727=CARTESIAN_POINT('Ctrl Pts',(-16.8482050523272,18.2489578333071,
-16.1511057276699));
#103728=CARTESIAN_POINT('Ctrl Pts',(-16.8237586672676,18.2973091739464,
-16.1477655338939));
#103729=CARTESIAN_POINT('Ctrl Pts',(-16.8041453398379,18.3394994849612,
-16.1448213375566));
#103730=CARTESIAN_POINT('Ctrl Pts',(-16.7578584182424,18.4483078538434,
-16.1372153721465));
#103731=CARTESIAN_POINT('Ctrl Pts',(-16.7331524756047,18.5156993492254,
-16.1324938667296));
#103732=CARTESIAN_POINT('Ctrl Pts',(-16.6793506439932,18.689269391624,-16.1204918437005));
#103733=CARTESIAN_POINT('Ctrl Pts',(-16.655020052626,18.7967143134445,-16.113215157046));
#103734=CARTESIAN_POINT('Ctrl Pts',(-16.6280926791828,18.9814003830941,
-16.1012114343839));
#103735=CARTESIAN_POINT('Ctrl Pts',(-16.6211610826707,19.057782449653,-16.0963862281508));
#103736=CARTESIAN_POINT('Ctrl Pts',(-16.617698500051,19.1533906761853,-16.0905240376858));
#103737=CARTESIAN_POINT('Ctrl Pts',(-16.6172662600462,19.1724100518565,
-16.0893664208595));
#103738=CARTESIAN_POINT('Ctrl Pts',(-16.6170109972927,19.2000265936093,
-16.0876974929599));
#103739=CARTESIAN_POINT('Ctrl Pts',(-16.6169838936139,19.208620517816,-16.0871798217261));
#103740=CARTESIAN_POINT('Ctrl Pts',(-16.6170280710807,19.2236697994176,
-16.0862761713489));
#103741=CARTESIAN_POINT('Ctrl Pts',(-16.6170765472014,19.2301250639966,
-16.0858894830808));
#103742=CARTESIAN_POINT('Ctrl Pts',(-16.6172278474771,19.2426457256806,
-16.085141219004));
#103743=CARTESIAN_POINT('Ctrl Pts',(-16.6173272165513,19.2487110943414,
-16.0847795388207));
#103744=CARTESIAN_POINT('Ctrl Pts',(-16.6176266400319,19.2631880670412,
-16.0839181418249));
#103745=CARTESIAN_POINT('Ctrl Pts',(-16.6178507746571,19.2715991114692,
-16.0834191823888));
#103746=CARTESIAN_POINT('Ctrl Pts',(-16.618836410441,19.301819683382,-16.0816316780201));
#103747=CARTESIAN_POINT('Ctrl Pts',(-16.6198849956165,19.3236189415175,
-16.080352107594));
#103748=CARTESIAN_POINT('Ctrl Pts',(-16.6332258364744,19.5333351579009,
-16.0681267730325));
#103749=CARTESIAN_POINT('Ctrl Pts',(-16.6702009845931,19.7188301038407,
-16.0580678304988));
#103750=CARTESIAN_POINT('Ctrl Pts',(-16.7338899023924,19.9047694489388,
-16.0473468765687));
#103751=CARTESIAN_POINT('Ctrl Pts',(-16.7365964021646,19.9125235685369,
-16.0468983949908));
#103752=CARTESIAN_POINT('Ctrl Pts',(-16.7635062156403,19.988201860216,-16.0425061094997));
#103753=CARTESIAN_POINT('Ctrl Pts',(-16.7911181414163,20.0548583904252,
-16.03851835394));
#103754=CARTESIAN_POINT('Ctrl Pts',(-16.8365787807688,20.1504801333401,
-16.0324474626111));
#103755=CARTESIAN_POINT('Ctrl Pts',(-16.8518108267229,20.1806359260491,
-16.0304791075487));
#103756=CARTESIAN_POINT('Ctrl Pts',(-16.8712146971588,20.2168695578073,
-16.028032312617));
#103757=CARTESIAN_POINT('Ctrl Pts',(-16.8747060574799,20.223308591068,-16.0275942967341));
#103758=CARTESIAN_POINT('Ctrl Pts',(-16.8802173408241,20.233348226445,-16.0269061294324));
#103759=CARTESIAN_POINT('Ctrl Pts',(-16.882214539102,20.2369613295415,-16.0266574054815));
#103760=CARTESIAN_POINT('Ctrl Pts',(-16.8859582051346,20.2436873995666,
-16.0261923566797));
#103761=CARTESIAN_POINT('Ctrl Pts',(-16.8877019816805,20.2468017994313,
-16.0259762041059));
#103762=CARTESIAN_POINT('Ctrl Pts',(-16.8916884439503,20.2538796040716,
-16.0254831153073));
#103763=CARTESIAN_POINT('Ctrl Pts',(-16.8939360379762,20.2578401754368,
-16.025205866663));
#103764=CARTESIAN_POINT('Ctrl Pts',(-16.8998091730102,20.2681120982282,
-16.024483415622));
#103765=CARTESIAN_POINT('Ctrl Pts',(-16.9034544805502,20.2744119971818,
-16.0240369841845));
#103766=CARTESIAN_POINT('Ctrl Pts',(-16.9267971713586,20.314277656614,-16.0211913093439));
#103767=CARTESIAN_POINT('Ctrl Pts',(-16.9473832047431,20.3473114176137,
-16.0187400319804));
#103768=CARTESIAN_POINT('Ctrl Pts',(-16.9758135989824,20.3902488851156,
-16.0154472396442));
#103769=CARTESIAN_POINT('Ctrl Pts',(-16.9828542120191,20.4006788522976,
-16.0146387986469));
#103770=CARTESIAN_POINT('Ctrl Pts',(-16.9904245042244,20.4116806759051,
-16.0137773451498));
#103771=CARTESIAN_POINT('Ctrl Pts',(-16.9908620922761,20.4123158742041,
-16.0137275775549));
#103772=CARTESIAN_POINT('Ctrl Pts',(-17.0042646762541,20.4317481854973,
-16.0122041174098));
#103773=CARTESIAN_POINT('Ctrl Pts',(-17.0175322919634,20.4503340862889,
-16.0107199756703));
#103774=CARTESIAN_POINT('Ctrl Pts',(-17.0582311857513,20.505439576628,-16.0062452323129));
#103775=CARTESIAN_POINT('Ctrl Pts',(-17.0865459466897,20.541289400095,-16.0032339605214));
#103776=CARTESIAN_POINT('Ctrl Pts',(-17.1865153883683,20.6597712945726,
-15.9929935655849));
#103777=CARTESIAN_POINT('Ctrl Pts',(-17.263408725544,20.7377650956525,-15.9857629846217));
#103778=CARTESIAN_POINT('Ctrl Pts',(-17.3875659455602,20.8455753095296,
-15.9751939953206));
#103779=CARTESIAN_POINT('Ctrl Pts',(-17.4305385328928,20.8800446754882,
-15.971707194325));
#103780=CARTESIAN_POINT('Ctrl Pts',(-17.5023719664899,20.9331953982135,
-15.9661529096575));
#103781=CARTESIAN_POINT('Ctrl Pts',(-17.5304269993849,20.9529175786369,
-15.9640470438692));
#103782=CARTESIAN_POINT('Ctrl Pts',(-17.5679391532657,20.9779487496927,
-15.9613116042486));
#103783=CARTESIAN_POINT('Ctrl Pts',(-17.5769741492196,20.9838781598675,
-15.9606587123239));
#103784=CARTESIAN_POINT('Ctrl Pts',(-17.591849766667,20.9934784490865,-15.9595933491927));
#103785=CARTESIAN_POINT('Ctrl Pts',(-17.5976635456929,20.9971903709641,
-15.9591793492999));
#103786=CARTESIAN_POINT('Ctrl Pts',(-17.6089545755137,21.004321913216,-15.958379849413));
#103787=CARTESIAN_POINT('Ctrl Pts',(-17.6144295268014,21.0077450148938,
-15.957994223246));
#103788=CARTESIAN_POINT('Ctrl Pts',(-17.627110153192,21.0155928528859,-15.9571057350838));
#103789=CARTESIAN_POINT('Ctrl Pts',(-17.6343268788482,21.019999592989,-15.9566035394799));
#103790=CARTESIAN_POINT('Ctrl Pts',(-17.6538130496318,21.031738709375,-15.955256670784));
#103791=CARTESIAN_POINT('Ctrl Pts',(-17.6661308039446,21.0389903420421,
-15.9544149408887));
#103792=CARTESIAN_POINT('Ctrl Pts',(-17.7800282815023,21.1044991766738,
-15.9467175539741));
#103793=CARTESIAN_POINT('Ctrl Pts',(-17.8862102169174,21.1543627927072,
-15.9401801184914));
#103794=CARTESIAN_POINT('Ctrl Pts',(-18.149351189169,21.2522374261536,-15.9248117443155));
#103795=CARTESIAN_POINT('Ctrl Pts',(-18.3087951046561,21.2913011832654,
-15.9161664957415));
#103796=CARTESIAN_POINT('Ctrl Pts',(-18.50235256656,21.3155234582328,-15.9049531343579));
#103797=CARTESIAN_POINT('Ctrl Pts',(-18.5336629100701,21.3187344072621,
-15.9031160160048));
#103798=CARTESIAN_POINT('Ctrl Pts',(-18.5721758821249,21.3218181655332,
-15.9008152056053));
#103799=CARTESIAN_POINT('Ctrl Pts',(-18.5793232595021,21.3223539437233,
-15.9003864797161));
#103800=CARTESIAN_POINT('Ctrl Pts',(-18.5905569754538,21.3231386929154,
-15.8997097260526));
#103801=CARTESIAN_POINT('Ctrl Pts',(-18.5946416269823,21.3234121289697,
-15.8994630491412));
#103802=CARTESIAN_POINT('Ctrl Pts',(-18.6022940386029,21.3239021074384,
-15.8989997354534));
#103803=CARTESIAN_POINT('Ctrl Pts',(-18.6058615626866,21.3241214626936,
-15.8987832581252));
#103804=CARTESIAN_POINT('Ctrl Pts',(-18.6140274890591,21.3246028033999,
-15.8982866560618));
#103805=CARTESIAN_POINT('Ctrl Pts',(-18.6186261878211,21.3248588165862,
-15.8980062011227));
#103806=CARTESIAN_POINT('Ctrl Pts',(-18.6328371777069,21.3256034424395,
-15.8971371701318));
#103807=CARTESIAN_POINT('Ctrl Pts',(-18.6424518363504,21.3260415033971,
-15.896545874289));
#103808=CARTESIAN_POINT('Ctrl Pts',(-18.7385987729991,21.3297653233294,
-15.8906017610589));
#103809=CARTESIAN_POINT('Ctrl Pts',(-18.8252432442561,21.3278039214104,
-15.8849959527821));
#103810=CARTESIAN_POINT('Ctrl Pts',(-19.0379878403697,21.3099019842061,
-15.8709783137679));
#103811=CARTESIAN_POINT('Ctrl Pts',(-19.1632592867183,21.2879059161919,
-15.8625169320018));
#103812=CARTESIAN_POINT('Ctrl Pts',(-19.3790107608838,21.2296555508022,
-15.8480526990988));
#103813=CARTESIAN_POINT('Ctrl Pts',(-19.4703935014274,21.1981432415498,
-15.8419580184891));
#103814=CARTESIAN_POINT('Ctrl Pts',(-19.5727827760602,21.1547968694471,
-15.8351790868987));
#103815=CARTESIAN_POINT('Ctrl Pts',(-19.5861890623735,21.1489568194085,
-15.8342923275355));
#103816=CARTESIAN_POINT('Ctrl Pts',(-19.6065883425571,21.1398178596174,
-15.8329440589035));
#103817=CARTESIAN_POINT('Ctrl Pts',(-19.6136253611061,21.1366188557751,
-15.8324791452786));
#103818=CARTESIAN_POINT('Ctrl Pts',(-19.6264196539959,21.1307178450611,
-15.8316341617966));
#103819=CARTESIAN_POINT('Ctrl Pts',(-19.632182550925,21.1280283122751,-15.8312536680764));
#103820=CARTESIAN_POINT('Ctrl Pts',(-19.6446241845002,21.1221534068775,
-15.8304324110532));
#103821=CARTESIAN_POINT('Ctrl Pts',(-19.6512985327573,21.1189588973426,
-15.8299919700129));
#103822=CARTESIAN_POINT('Ctrl Pts',(-19.669415281113,21.1101707307961,-15.8287966965718));
#103823=CARTESIAN_POINT('Ctrl Pts',(-19.680824287376,21.1045086459663,-15.8280442518747));
#103824=CARTESIAN_POINT('Ctrl Pts',(-19.7368646365838,21.0760636656641,
-15.8243487489689));
#103825=CARTESIAN_POINT('Ctrl Pts',(-19.7807305047689,21.0518030280639,
-15.8214580571016));
#103826=CARTESIAN_POINT('Ctrl Pts',(-19.9725201961351,20.9366560268146,
-15.8087586900135));
#103827=CARTESIAN_POINT('Ctrl Pts',(-20.1097822015029,20.8293461344433,
-15.7995652052348));
#103828=CARTESIAN_POINT('Ctrl Pts',(-20.2767028284257,20.6620992837642,
-15.7865789601383));
#103829=CARTESIAN_POINT('Ctrl Pts',(-20.3190029595376,20.6157724433836,
-15.7830864700019));
#103830=CARTESIAN_POINT('Ctrl Pts',(-20.3790002882388,20.5438989080495,
-15.7777012142349));
#103831=CARTESIAN_POINT('Ctrl Pts',(-20.3982951617297,20.5197271812692,
-15.7758951897647));
#103832=CARTESIAN_POINT('Ctrl Pts',(-20.4213765010813,20.489475794707,-15.773629017466));
#103833=CARTESIAN_POINT('Ctrl Pts',(-20.4256717671369,20.4837868804455,
-15.7732026023112));
#103834=CARTESIAN_POINT('Ctrl Pts',(-20.4323832435559,20.4748038007864,
-15.772528688803));
#103835=CARTESIAN_POINT('Ctrl Pts',(-20.4348188352532,20.471524088573,-15.7722825225411));
#103836=CARTESIAN_POINT('Ctrl Pts',(-20.4393684431166,20.4653604980719,
-15.7718196309149));
#103837=CARTESIAN_POINT('Ctrl Pts',(-20.4414846510052,20.4624783065653,
-15.7716030617624));
#103838=CARTESIAN_POINT('Ctrl Pts',(-20.4463180504728,20.4558603268095,
-15.7711055340077));
#103839=CARTESIAN_POINT('Ctrl Pts',(-20.4490303153541,20.4521210076871,
-15.7708242405577));
#103840=CARTESIAN_POINT('Ctrl Pts',(-20.4573967032765,20.4405067253994,
-15.7699500730901));
#103841=CARTESIAN_POINT('Ctrl Pts',(-20.4630088935388,20.4326019083675,
-15.7693544335711));
#103842=CARTESIAN_POINT('Ctrl Pts',(-20.5258583159912,20.3427772533996,
-15.762581057254));
#103843=CARTESIAN_POINT('Ctrl Pts',(-20.5772738099576,20.256950713446,-15.7560681325924));
#103844=CARTESIAN_POINT('Ctrl Pts',(-20.6995936298735,20.0155355212111,
-15.7382366497741));
#103845=CARTESIAN_POINT('Ctrl Pts',(-20.7580649026369,19.8544399609954,
-15.7269007947659));
#103846=CARTESIAN_POINT('Ctrl Pts',(-20.8065479238249,19.6448237985732,
-15.7134188741454));
#103847=CARTESIAN_POINT('Ctrl Pts',(-20.8151860530158,19.6012858729815,
-15.7106796434028));
#103848=CARTESIAN_POINT('Ctrl Pts',(-20.8243855575939,19.5458388959596,
-15.7072653515632));
#103849=CARTESIAN_POINT('Ctrl Pts',(-20.8262235205536,19.5341557125939,
-15.7065500432523));
#103850=CARTESIAN_POINT('Ctrl Pts',(-20.8290114867026,19.5154119083165,
-15.7054088837522));
#103851=CARTESIAN_POINT('Ctrl Pts',(-20.8300239034832,19.5083609545634,
-15.7049810632564));
#103852=CARTESIAN_POINT('Ctrl Pts',(-20.8318772340356,19.4949735307227,
-15.7041714885603));
#103853=CARTESIAN_POINT('Ctrl Pts',(-20.8327250735324,19.4886381140026,
-15.7037895194621));
#103854=CARTESIAN_POINT('Ctrl Pts',(-20.8345859303437,19.47423720362,-15.7029238434145));
#103855=CARTESIAN_POINT('Ctrl Pts',(-20.8355812167359,19.4661694895691,
-15.7024407011398));
#103856=CARTESIAN_POINT('Ctrl Pts',(-20.8380346046374,19.4452937228268,
-15.7011951507269));
#103857=CARTESIAN_POINT('Ctrl Pts',(-20.8394222487898,19.4324776091554,
-15.7004349637519));
#103858=CARTESIAN_POINT('Ctrl Pts',(-20.8476032826776,19.3498752888383,
-15.6955629874776));
#103859=CARTESIAN_POINT('Ctrl Pts',(-20.8510436184249,19.2797966553481,
-15.6915583274132));
#103860=CARTESIAN_POINT('Ctrl Pts',(-20.8508787727055,19.0172834305071,
-15.6768593416721));
#103861=CARTESIAN_POINT('Ctrl Pts',(-20.8245352158017,18.8258343963927,
-15.6668250131367));
#103862=CARTESIAN_POINT('Ctrl Pts',(-20.7592947702424,18.5926573079251,
-15.6531662906187));
#103863=CARTESIAN_POINT('Ctrl Pts',(-20.7441979123084,18.5452146740884,
-15.6503027919625));
#103864=CARTESIAN_POINT('Ctrl Pts',(-20.7258385779948,18.4938592559299,
-15.6470652940501));
#103865=CARTESIAN_POINT('Ctrl Pts',(-20.7242171643571,18.4893716987585,
-15.6467812224719));
#103866=CARTESIAN_POINT('Ctrl Pts',(-20.7225806137986,18.4848897174503,
-15.646496294977));
#103867=CARTESIAN_POINT('Origin',(-18.734,19.211,0.));
#103868=CARTESIAN_POINT('',(-20.7225806190038,18.4848897317057,-14.8438386123028));
#103869=CARTESIAN_POINT('',(-20.7193263794245,18.4860708438863,-15.0663814102382));
#103870=CARTESIAN_POINT('',(-20.7225806137986,18.4848897174502,0.));
#103871=CARTESIAN_POINT('',(-20.8523540121835,19.212740575366,-15.110942953294));
#103872=CARTESIAN_POINT('Ctrl Pts',(-20.7193263794245,18.4860708438863,
-15.0663814102382));
#103873=CARTESIAN_POINT('Ctrl Pts',(-20.8041092769325,18.7190474195728,
-15.0812352579235));
#103874=CARTESIAN_POINT('Ctrl Pts',(-20.8501557500904,18.9662442220235,
-15.0960891056087));
#103875=CARTESIAN_POINT('Ctrl Pts',(-20.8523540121835,19.212740575366,-15.110942953294));
#103876=CARTESIAN_POINT('Ctrl Pts',(-20.8509992391722,19.2127948104318,
-15.1101643277519));
#103877=CARTESIAN_POINT('Ctrl Pts',(-20.8509308762891,19.293429605496,-15.1145734088296));
#103878=CARTESIAN_POINT('Ctrl Pts',(-20.8462555791837,19.3739894416571,
-15.1190372239295));
#103879=CARTESIAN_POINT('Ctrl Pts',(-20.8342736513811,19.4776506928941,
-15.125070444969));
#103880=CARTESIAN_POINT('Ctrl Pts',(-20.831153212252,19.5011728849275,-15.1264590656482));
#103881=CARTESIAN_POINT('Ctrl Pts',(-20.8267556721879,19.5305280666389,
-15.128222132077));
#103882=CARTESIAN_POINT('Ctrl Pts',(-20.8258482444011,19.5364157484879,
-15.1285772658009));
#103883=CARTESIAN_POINT('Ctrl Pts',(-20.8242835005995,19.5462912490265,
-15.129175609063));
#103884=CARTESIAN_POINT('Ctrl Pts',(-20.8236395868589,19.5502811974942,
-15.1294180879065));
#103885=CARTESIAN_POINT('Ctrl Pts',(-20.822439937094,19.5575817335751,-15.1298631422263));
#103886=CARTESIAN_POINT('Ctrl Pts',(-20.821887742758,19.5608929010099,-15.1300655186597));
#103887=CARTESIAN_POINT('Ctrl Pts',(-20.8207312363697,19.5677275251417,
-15.1304843497052));
#103888=CARTESIAN_POINT('Ctrl Pts',(-20.8201258792699,19.5712507393469,
-15.130700865115));
#103889=CARTESIAN_POINT('Ctrl Pts',(-20.8187191843601,19.5793153386286,
-15.1311978541401));
#103890=CARTESIAN_POINT('Ctrl Pts',(-20.8179119319051,19.5838556361952,
-15.1314786599025));
#103891=CARTESIAN_POINT('Ctrl Pts',(-20.8153688766512,19.5978924881345,
-15.1323498378207));
#103892=CARTESIAN_POINT('Ctrl Pts',(-20.8135829728089,19.6073796780452,
-15.1329429488265));
#103893=CARTESIAN_POINT('Ctrl Pts',(-20.7944801201428,19.7051749508872,
-15.1390989358417));
#103894=CARTESIAN_POINT('Ctrl Pts',(-20.7716158268014,19.7922961060446,
-15.1449346741224));
#103895=CARTESIAN_POINT('Ctrl Pts',(-20.7285347464531,19.9221351934489,
-15.1539258486894));
#103896=CARTESIAN_POINT('Ctrl Pts',(-20.7123161216645,19.9660810243259,
-15.1570231572921));
#103897=CARTESIAN_POINT('Ctrl Pts',(-20.6795753796455,20.0464781316713,
-15.1627587620049));
#103898=CARTESIAN_POINT('Ctrl Pts',(-20.6634510471132,20.0830699643245,
-15.1653968831636));
#103899=CARTESIAN_POINT('Ctrl Pts',(-20.6009607306979,20.2146515176478,
-15.1749557043506));
#103900=CARTESIAN_POINT('Ctrl Pts',(-20.5485314129769,20.3066001941314,
-15.1817659660048));
#103901=CARTESIAN_POINT('Ctrl Pts',(-20.4701931586325,20.4228204414318,
-15.190478866321));
#103902=CARTESIAN_POINT('Ctrl Pts',(-20.4502456482645,20.45090990002,-15.1925946173668));
#103903=CARTESIAN_POINT('Ctrl Pts',(-20.4231395493703,20.487171523434,-15.1953408209963));
#103904=CARTESIAN_POINT('Ctrl Pts',(-20.4165920234465,20.4957919146388,
-15.195994821804));
#103905=CARTESIAN_POINT('Ctrl Pts',(-20.4057621089003,20.5098256554026,
-15.1970615305458));
#103906=CARTESIAN_POINT('Ctrl Pts',(-20.4015189162918,20.5152688746768,
-15.197475774627));
#103907=CARTESIAN_POINT('Ctrl Pts',(-20.3932555401393,20.5257629913607,
-15.1982754261272));
#103908=CARTESIAN_POINT('Ctrl Pts',(-20.3892387286754,20.5308164355138,
-15.1986609613961));
#103909=CARTESIAN_POINT('Ctrl Pts',(-20.3799132798929,20.5424389988433,
-15.1995487834451));
#103910=CARTESIAN_POINT('Ctrl Pts',(-20.3745882971521,20.5489949084246,
-15.2000504070404));
#103911=CARTESIAN_POINT('Ctrl Pts',(-20.3601678655803,20.5665332554568,
-15.2013947294498));
#103912=CARTESIAN_POINT('Ctrl Pts',(-20.3510003542833,20.5774560742156,
-15.2022345026572));
#103913=CARTESIAN_POINT('Ctrl Pts',(-20.2485615925972,20.6970341414247,
-15.211459206279));
#103914=CARTESIAN_POINT('Ctrl Pts',(-20.1446034879664,20.7960551416562,
-15.2193503669587));
#103915=CARTESIAN_POINT('Ctrl Pts',(-19.9525871115183,20.944980926329,-15.2325685024283));
#103916=CARTESIAN_POINT('Ctrl Pts',(-19.8695239176921,21.0004770268959,
-15.2379407463332));
#103917=CARTESIAN_POINT('Ctrl Pts',(-19.7435196494029,21.0723464026377,
-15.2460221682943));
#103918=CARTESIAN_POINT('Ctrl Pts',(-19.7034698356571,21.0935164202032,
-15.2485825476238));
#103919=CARTESIAN_POINT('Ctrl Pts',(-19.6404725697104,21.1242726983585,
-15.25264384672));
#103920=CARTESIAN_POINT('Ctrl Pts',(-19.6179818126113,21.1347673901187,
-15.2541002780795));
#103921=CARTESIAN_POINT('Ctrl Pts',(-19.5892751475924,21.1475528931052,
-15.2559738092091));
#103922=CARTESIAN_POINT('Ctrl Pts',(-19.5832249218171,21.1502136848249,
-15.2563694856048));
#103923=CARTESIAN_POINT('Ctrl Pts',(-19.5740558157435,21.1541949714397,
-15.2569705007484));
#103924=CARTESIAN_POINT('Ctrl Pts',(-19.5709459972217,21.1555364146649,
-15.2571745797304));
#103925=CARTESIAN_POINT('Ctrl Pts',(-19.5645603854714,21.1582727396786,
-15.2575941419284));
#103926=CARTESIAN_POINT('Ctrl Pts',(-19.5612843186643,21.1596668089167,
-15.257809672999));
#103927=CARTESIAN_POINT('Ctrl Pts',(-19.5539356860413,21.1627720113518,
-15.2582937606435));
#103928=CARTESIAN_POINT('Ctrl Pts',(-19.5498613024546,21.1644786530387,
-15.2585625825862));
#103929=CARTESIAN_POINT('Ctrl Pts',(-19.5394715451773,21.1687924484995,
-15.259249105988));
#103930=CARTESIAN_POINT('Ctrl Pts',(-19.5331488917613,21.1713817810249,
-15.2596678465849));
#103931=CARTESIAN_POINT('Ctrl Pts',(-19.4970328859625,21.1859687097063,
-15.2620647569134));
#103932=CARTESIAN_POINT('Ctrl Pts',(-19.4669837927748,21.1973169663692,
-15.2640783175986));
#103933=CARTESIAN_POINT('Ctrl Pts',(-19.2681647179833,21.2672768294484,
-15.2774734486702));
#103934=CARTESIAN_POINT('Ctrl Pts',(-19.0928126952863,21.3050066048381,
-15.2895530637602));
#103935=CARTESIAN_POINT('Ctrl Pts',(-18.8223031740019,21.328193932115,-15.3071745412507));
#103936=CARTESIAN_POINT('Ctrl Pts',(-18.7293755047119,21.3300304739467,
-15.3130657906812));
#103937=CARTESIAN_POINT('Ctrl Pts',(-18.6155530486077,21.3247889952998,
-15.320062630398));
#103938=CARTESIAN_POINT('Ctrl Pts',(-18.5945049993098,21.3235043886848,
-15.3213476054317));
#103939=CARTESIAN_POINT('Ctrl Pts',(-18.5645469881221,21.3212262721467,
-15.3231644411897));
#103940=CARTESIAN_POINT('Ctrl Pts',(-18.5556192325636,21.3204903528001,
-15.323704344491));
#103941=CARTESIAN_POINT('Ctrl Pts',(-18.5402049144886,21.3191211861481,
-15.3246339506053));
#103942=CARTESIAN_POINT('Ctrl Pts',(-18.5337161622062,21.3185146159511,
-15.3250244863652));
#103943=CARTESIAN_POINT('Ctrl Pts',(-18.5212831731226,21.3172944381121,
-15.3257713111947));
#103944=CARTESIAN_POINT('Ctrl Pts',(-18.5153385403187,21.3166856070259,
-15.3261277465956));
#103945=CARTESIAN_POINT('Ctrl Pts',(-18.4998558430929,21.315033643864,-15.3270544325623));
#103946=CARTESIAN_POINT('Ctrl Pts',(-18.4903220825626,21.3139508168013,
-15.3276234288962));
#103947=CARTESIAN_POINT('Ctrl Pts',(-18.4576767400547,21.310018034307,-15.3295664486316));
#103948=CARTESIAN_POINT('Ctrl Pts',(-18.4346044783592,21.3068515303342,
-15.3309305008786));
#103949=CARTESIAN_POINT('Ctrl Pts',(-18.2424793265693,21.2772462057837,
-15.3422230489624));
#103950=CARTESIAN_POINT('Ctrl Pts',(-18.0771536862297,21.2307835874841,
-15.3514435394357));
#103951=CARTESIAN_POINT('Ctrl Pts',(-17.8360461671051,21.1302412468535,
-15.3656482801688));
#103952=CARTESIAN_POINT('Ctrl Pts',(-17.755186825856,21.0902898235673,-15.3705714861155));
#103953=CARTESIAN_POINT('Ctrl Pts',(-17.6436818181249,21.0260440874248,
-15.3779131172016));
#103954=CARTESIAN_POINT('Ctrl Pts',(-17.6107737720088,21.0058652304271,
-15.3801538389643));
#103955=CARTESIAN_POINT('Ctrl Pts',(-17.5720572298016,20.9806428997978,
-15.3829028032305));
#103956=CARTESIAN_POINT('Ctrl Pts',(-17.56569901276,20.9764517249826,-15.3833579837891));
#103957=CARTESIAN_POINT('Ctrl Pts',(-17.5558763608704,20.9699005832118,
-15.3840672155997));
#103958=CARTESIAN_POINT('Ctrl Pts',(-17.5523960148206,20.9675644287095,
-15.3843196930339));
#103959=CARTESIAN_POINT('Ctrl Pts',(-17.5459702208747,20.9632234272667,
-15.3847880835773));
#103960=CARTESIAN_POINT('Ctrl Pts',(-17.5430228872354,20.9612214749711,
-15.385003801407));
#103961=CARTESIAN_POINT('Ctrl Pts',(-17.5363909910637,20.9566923051825,
-15.3854911788369));
#103962=CARTESIAN_POINT('Ctrl Pts',(-17.5327093894604,20.9541608734829,
-15.3857631212966));
#103963=CARTESIAN_POINT('Ctrl Pts',(-17.5219242170672,20.946694705068,-15.3865637700496));
#103964=CARTESIAN_POINT('Ctrl Pts',(-17.5148429428926,20.9417281349256,
-15.3870945721637));
#103965=CARTESIAN_POINT('Ctrl Pts',(-17.4656337775459,20.906762609763,-15.3908179403918));
#103966=CARTESIAN_POINT('Ctrl Pts',(-17.4245905926597,20.8752745424576,
-15.3941017659741));
#103967=CARTESIAN_POINT('Ctrl Pts',(-17.36792480951,20.8284065797107,-15.3988492516395));
#103968=CARTESIAN_POINT('Ctrl Pts',(-17.3513209985764,20.8142355420827,
-15.4002679591068));
#103969=CARTESIAN_POINT('Ctrl Pts',(-17.2968372836858,20.7662587725617,
-15.4050090025746));
#103970=CARTESIAN_POINT('Ctrl Pts',(-17.2599550183476,20.7313478792839,
-15.4083593014268));
#103971=CARTESIAN_POINT('Ctrl Pts',(-17.1593371371747,20.6290019140577,
-15.4178426493096));
#103972=CARTESIAN_POINT('Ctrl Pts',(-17.0987236173138,20.5586518900657,
-15.4239710749371));
#103973=CARTESIAN_POINT('Ctrl Pts',(-17.0051196442341,20.434359884108,-15.4340313087819));
#103974=CARTESIAN_POINT('Ctrl Pts',(-16.9695724088146,20.382508919724,-15.4380304668877));
#103975=CARTESIAN_POINT('Ctrl Pts',(-16.9232015395132,20.3079597301001,
-15.4435029450439));
#103976=CARTESIAN_POINT('Ctrl Pts',(-16.9103965770584,20.2865381687643,
-15.4450452248955));
#103977=CARTESIAN_POINT('Ctrl Pts',(-16.8886448095702,20.248643640418,-15.4477217150988));
#103978=CARTESIAN_POINT('Ctrl Pts',(-16.8795326393471,20.2322692823418,
-15.4488617409194));
#103979=CARTESIAN_POINT('Ctrl Pts',(-16.8665848612835,20.2082575677118,
-15.4505101004298));
#103980=CARTESIAN_POINT('Ctrl Pts',(-16.86257638092,20.2007149074131,-15.4510245765895));
#103981=CARTESIAN_POINT('Ctrl Pts',(-16.8556225263117,20.1874367020347,
-15.4519245384563));
#103982=CARTESIAN_POINT('Ctrl Pts',(-16.8526575199355,20.1817116157084,
-15.452310715752));
#103983=CARTESIAN_POINT('Ctrl Pts',(-16.8469466664498,20.1705601594194,
-15.4530593626258));
#103984=CARTESIAN_POINT('Ctrl Pts',(-16.8441979596499,20.1651353324785,
-15.4534219301234));
#103985=CARTESIAN_POINT('Ctrl Pts',(-16.8376761363859,20.1521251649403,
-15.4542876228486));
#103986=CARTESIAN_POINT('Ctrl Pts',(-16.8339250828848,20.1445288342177,
-15.45478997313));
#103987=CARTESIAN_POINT('Ctrl Pts',(-16.8205146696674,20.1169554440092,
-15.4566023922238));
#103988=CARTESIAN_POINT('Ctrl Pts',(-16.8111237292017,20.0968489024758,
-15.4579031508943));
#103989=CARTESIAN_POINT('Ctrl Pts',(-16.7265023657435,19.9079803521537,
-15.4699389098787));
#103990=CARTESIAN_POINT('Ctrl Pts',(-16.6733539663025,19.7302035952761,
-15.4798262352747));
#103991=CARTESIAN_POINT('Ctrl Pts',(-16.6311238172708,19.468118820722,-15.4942953529183));
#103992=CARTESIAN_POINT('Ctrl Pts',(-16.6228541218484,19.3878032036988,
-15.4987306268947));
#103993=CARTESIAN_POINT('Ctrl Pts',(-16.6175435583974,19.271081242806,-15.5054131239299));
#103994=CARTESIAN_POINT('Ctrl Pts',(-16.6168260371573,19.2349099032179,
-15.5075170520817));
#103995=CARTESIAN_POINT('Ctrl Pts',(-16.6170787854484,19.1912655893302,
-15.5101143634216));
#103996=CARTESIAN_POINT('Ctrl Pts',(-16.617161662064,19.1837911255862,-15.5105612543756));
#103997=CARTESIAN_POINT('Ctrl Pts',(-16.617352293182,19.1721567113908,-15.5112603173794));
#103998=CARTESIAN_POINT('Ctrl Pts',(-16.6174327329262,19.1679962895193,
-15.5115109870723));
#103999=CARTESIAN_POINT('Ctrl Pts',(-16.6176048767735,19.1602713423011,
-15.5119777441079));
#104000=CARTESIAN_POINT('Ctrl Pts',(-16.6176933203464,19.1567068017264,
-15.5121936471735));
#104001=CARTESIAN_POINT('Ctrl Pts',(-16.6179139712989,19.1486362213743,
-15.5126836657305));
#104002=CARTESIAN_POINT('Ctrl Pts',(-16.6180515657088,19.1441303933021,
-15.5129580778639));
#104003=CARTESIAN_POINT('Ctrl Pts',(-16.6185014370032,19.1307946699384,
-15.5137726427061));
#104004=CARTESIAN_POINT('Ctrl Pts',(-16.6188545976371,19.1219663792137,
-15.5143149995884));
#104005=CARTESIAN_POINT('Ctrl Pts',(-16.6218674308755,19.0568591049924,
-15.5183364794709));
#104006=CARTESIAN_POINT('Ctrl Pts',(-16.626717417804,19.0007089470725,-15.5219238152531));
#104007=CARTESIAN_POINT('Ctrl Pts',(-16.6548174068893,18.7789918878224,
-15.5363951828686));
#104008=CARTESIAN_POINT('Ctrl Pts',(-16.6954012390558,18.6162278000266,
-15.5476444985705));
#104009=CARTESIAN_POINT('Ctrl Pts',(-16.7754762364667,18.4052096757778,
-15.5621909727667));
#104010=CARTESIAN_POINT('Ctrl Pts',(-16.7984984579841,18.3513790770242,
-15.5659051320982));
#104011=CARTESIAN_POINT('Ctrl Pts',(-16.8391656876571,18.2662378032368,
-15.5717775253957));
#104012=CARTESIAN_POINT('Ctrl Pts',(-16.8554267749238,18.2343037504129,
-15.5739798485299));
#104013=CARTESIAN_POINT('Ctrl Pts',(-16.877720624992,18.1931412449418,-15.5768200697672));
#104014=CARTESIAN_POINT('Ctrl Pts',(-16.8830249343894,18.1835269458855,
-15.5774835779558));
#104015=CARTESIAN_POINT('Ctrl Pts',(-16.8918014861631,18.1679076068336,
-15.5785618268884));
#104016=CARTESIAN_POINT('Ctrl Pts',(-16.8952288134719,18.161877685663,-15.5789781682825));
#104017=CARTESIAN_POINT('Ctrl Pts',(-16.901896685097,18.1502795149001,-15.5797791683223));
#104018=CARTESIAN_POINT('Ctrl Pts',(-16.905133130337,18.1447090085468,-15.5801639690235));
#104019=CARTESIAN_POINT('Ctrl Pts',(-16.9126301840842,18.1319397765896,
-15.5810462905161));
#104020=CARTESIAN_POINT('Ctrl Pts',(-16.9169081493606,18.1247513261319,
-15.581543174618));
#104021=CARTESIAN_POINT('Ctrl Pts',(-16.928449973859,18.1056160914496,-15.5828664627004));
#104022=CARTESIAN_POINT('Ctrl Pts',(-16.9357898428663,18.0937154673312,
-15.5836900843806));
#104023=CARTESIAN_POINT('Ctrl Pts',(-16.9968414899234,17.9968885552311,
-15.5903986846492));
#104024=CARTESIAN_POINT('Ctrl Pts',(-17.0564229172238,17.9158069053196,
-15.5960544393299));
#104025=CARTESIAN_POINT('Ctrl Pts',(-17.2326520132677,17.7086535594027,
-15.6110382220004));
#104026=CARTESIAN_POINT('Ctrl Pts',(-17.3591999744398,17.5920485162329,
-15.6200522704073));
#104027=CARTESIAN_POINT('Ctrl Pts',(-17.5308011486323,17.4687046231591,
-15.6320928078035));
#104028=CARTESIAN_POINT('Ctrl Pts',(-17.5638458944849,17.4463415167844,
-15.6344066297458));
#104029=CARTESIAN_POINT('Ctrl Pts',(-17.603984818917,17.4208006346096,-15.6372365700519));
#104030=CARTESIAN_POINT('Ctrl Pts',(-17.6104918134872,17.4167097703938,
-15.6376959303295));
#104031=CARTESIAN_POINT('Ctrl Pts',(-17.6205946336153,17.4104347583439,
-15.6384102861626));
#104032=CARTESIAN_POINT('Ctrl Pts',(-17.6241750129557,17.4082256944421,
-15.6386636713128));
#104033=CARTESIAN_POINT('Ctrl Pts',(-17.6307988481412,17.4041660547059,
-15.6391328976393));
#104034=CARTESIAN_POINT('Ctrl Pts',(-17.6338403990617,17.4023124815941,
-15.6393485380588));
#104035=CARTESIAN_POINT('Ctrl Pts',(-17.6406913639609,17.3981610612338,
-15.6398346599955));
#104036=CARTESIAN_POINT('Ctrl Pts',(-17.6445033266221,17.3958675559601,
-15.6401054177427));
#104037=CARTESIAN_POINT('Ctrl Pts',(-17.6542753583027,17.3900299889312,
-15.6408001508312));
#104038=CARTESIAN_POINT('Ctrl Pts',(-17.6602456092922,17.3865031958119,
-15.6412252074449));
#104039=CARTESIAN_POINT('Ctrl Pts',(-17.6952194998654,17.3660742645413,
-15.6437182468139));
#104040=CARTESIAN_POINT('Ctrl Pts',(-17.7246028171321,17.3498355978042,
-15.6458249132462));
#104041=CARTESIAN_POINT('Ctrl Pts',(-17.7705504057268,17.3258507941892,
-15.6491234501822));
#104042=CARTESIAN_POINT('Ctrl Pts',(-17.7868513488715,17.3176083222549,
-15.6502945011103));
#104043=CARTESIAN_POINT('Ctrl Pts',(-17.8254406850437,17.2987188928704,
-15.6530653765505));
#104044=CARTESIAN_POINT('Ctrl Pts',(-17.847812677376,17.2882490997966,-15.6546707154741));
#104045=CARTESIAN_POINT('Ctrl Pts',(-17.9113738267982,17.2598483010576,
-15.6592195973515));
#104046=CARTESIAN_POINT('Ctrl Pts',(-17.952957538278,17.2428335266386,-15.6621813712387));
#104047=CARTESIAN_POINT('Ctrl Pts',(-18.097516943307,17.1889875012088,-15.6723715840893));
#104048=CARTESIAN_POINT('Ctrl Pts',(-18.2027950029202,17.1588133748115,
-15.6796016161337));
#104049=CARTESIAN_POINT('Ctrl Pts',(-18.3638784493342,17.1258788673889,
-15.690169452627));
#104050=CARTESIAN_POINT('Ctrl Pts',(-18.4182309640556,17.1169582537551,
-15.6936556535534));
#104051=CARTESIAN_POINT('Ctrl Pts',(-18.5068944721206,17.1059376735066,
-15.6992090942802));
#104052=CARTESIAN_POINT('Ctrl Pts',(-18.5410147457956,17.1025358132481,
-15.7013147016574));
#104053=CARTESIAN_POINT('Ctrl Pts',(-18.5859799021831,17.09915345664,-15.7040498598085));
#104054=CARTESIAN_POINT('Ctrl Pts',(-18.5967617721105,17.0984253983241,
-15.7047027226738));
#104055=CARTESIAN_POINT('Ctrl Pts',(-18.6144340885846,17.0973679202973,
-15.7057680505384));
#104056=CARTESIAN_POINT('Ctrl Pts',(-18.6213213088794,17.0969895719652,
-15.7061820440289));
#104057=CARTESIAN_POINT('Ctrl Pts',(-18.6346591959332,17.0963222238912,
-15.7069815399475));
#104058=CARTESIAN_POINT('Ctrl Pts',(-18.6411095693041,17.096029063691,-15.7073671685044));
#104059=CARTESIAN_POINT('Ctrl Pts',(-18.6560100722666,17.0954201567498,
-15.7082556741727));
#104060=CARTESIAN_POINT('Ctrl Pts',(-18.6644609903024,17.0951255161779,
-15.7087578848085));
#104061=CARTESIAN_POINT('Ctrl Pts',(-18.6872016752728,17.0944690558154,
-15.7101048204557));
#104062=CARTESIAN_POINT('Ctrl Pts',(-18.701493872113,17.094201311541,-15.7109466018071));
#104063=CARTESIAN_POINT('Ctrl Pts',(-18.8329520761609,17.0930703659304,
-15.7186481019253));
#104064=CARTESIAN_POINT('Ctrl Pts',(-18.9500047665745,17.1017905072283,
-15.7251891916009));
#104065=CARTESIAN_POINT('Ctrl Pts',(-19.2275947590501,17.1458348607374,
-15.740574114917));
#104066=CARTESIAN_POINT('Ctrl Pts',(-19.385891996478,17.1902161640664,-15.7492315332679));
#104067=CARTESIAN_POINT('Ctrl Pts',(-19.5663317158214,17.2642369783433,
-15.7604463348995));
#104068=CARTESIAN_POINT('Ctrl Pts',(-19.5949289438936,17.2767137056503,
-15.7622678532734));
#104069=CARTESIAN_POINT('Ctrl Pts',(-19.6297251036186,17.2928194474207,
-15.764551288169));
#104070=CARTESIAN_POINT('Ctrl Pts',(-19.6361965560468,17.2958547145226,
-15.7649788602261));
#104071=CARTESIAN_POINT('Ctrl Pts',(-19.6463460677891,17.3006779389942,
-15.7656541957518));
#104072=CARTESIAN_POINT('Ctrl Pts',(-19.6500345982701,17.3024439127191,
-15.7659006177446));
#104073=CARTESIAN_POINT('Ctrl Pts',(-19.6569379755142,17.3057736947616,
-15.7663637201713));
#104074=CARTESIAN_POINT('Ctrl Pts',(-19.6601539858711,17.3073349626055,
-15.7665802427708));
#104075=CARTESIAN_POINT('Ctrl Pts',(-19.667510377405,17.3109293035762,-15.7670773043563));
#104076=CARTESIAN_POINT('Ctrl Pts',(-19.67164806648,17.3129677614361,-15.7673581758534));
#104077=CARTESIAN_POINT('Ctrl Pts',(-19.6824718143487,17.3183441773327,
-15.7680962340777));
#104078=CARTESIAN_POINT('Ctrl Pts',(-19.6891468506394,17.3217040105861,
-15.7685547368358));
#104079=CARTESIAN_POINT('Ctrl Pts',(-19.7338277385277,17.34449112986,-15.7716456005952));
#104080=CARTESIAN_POINT('Ctrl Pts',(-19.7712535947661,17.3650272804875,
-15.7743405593274));
#104081=CARTESIAN_POINT('Ctrl Pts',(-19.8142373262288,17.3903330337849,
-15.7775396770944));
#104082=CARTESIAN_POINT('Ctrl Pts',(-19.8204257247185,17.3940189804479,
-15.7780028388094));
#104083=CARTESIAN_POINT('Ctrl Pts',(-19.9612667857937,17.4788837828544,
-15.7886010872205));
#104084=CARTESIAN_POINT('Ctrl Pts',(-20.0864795944153,17.5747810010984,
-15.7991743407422));
#104085=CARTESIAN_POINT('Ctrl Pts',(-20.2683631241046,17.7493510044569,
-15.8155534689647));
#104086=CARTESIAN_POINT('Ctrl Pts',(-20.3323175753978,17.8195715623013,
-15.8215790948944));
#104087=CARTESIAN_POINT('Ctrl Pts',(-20.4046232446554,17.9105531873314,
-15.828717173166));
#104088=CARTESIAN_POINT('Ctrl Pts',(-20.4176410421793,17.9274514689708,
-15.8300172200694));
#104089=CARTESIAN_POINT('Ctrl Pts',(-20.4357852628147,17.9517554224721,
-15.8318514462579));
#104090=CARTESIAN_POINT('Ctrl Pts',(-20.441122932127,17.959001084153,-15.832393879567));
#104091=CARTESIAN_POINT('Ctrl Pts',(-20.4502504309324,17.9715581794512,
-15.8333264665723));
#104092=CARTESIAN_POINT('Ctrl Pts',(-20.4540621751043,17.9768534594887,
-15.8337174675283));
#104093=CARTESIAN_POINT('Ctrl Pts',(-20.4613129506172,17.9870250924257,
-15.8344642456815));
#104094=CARTESIAN_POINT('Ctrl Pts',(-20.4647559588594,17.991898521149,-15.8348201737037));
#104095=CARTESIAN_POINT('Ctrl Pts',(-20.4736538394492,18.004606757036,-15.8357435117079));
#104096=CARTESIAN_POINT('Ctrl Pts',(-20.4790764406837,18.0124640770974,
-15.8363096855944));
#104097=CARTESIAN_POINT('Ctrl Pts',(-20.497378061547,18.0393705632119,-15.8382327433023));
#104098=CARTESIAN_POINT('Ctrl Pts',(-20.5100000812378,18.0585931718865,
-15.8395799350522));
#104099=CARTESIAN_POINT('Ctrl Pts',(-20.603475270823,18.2061350947592,-15.84972915068));
#104100=CARTESIAN_POINT('Ctrl Pts',(-20.6706038614521,18.342542247002,-15.8579870587477));
#104101=CARTESIAN_POINT('Ctrl Pts',(-20.722580613579,18.4848897168488,-15.866216451952));
#104102=CARTESIAN_POINT('',(-20.8509997481126,19.2099672893213,-14.890777245922));
#104103=CARTESIAN_POINT('Ctrl Pts',(-20.7225806137986,18.4848897174503,
-15.646496294977));
#104104=CARTESIAN_POINT('Ctrl Pts',(-20.7215382221587,18.4820349447569,
-15.6463148120176));
#104105=CARTESIAN_POINT('Ctrl Pts',(-20.7204896894983,18.4791824341809,
-15.6461329818143));
#104106=CARTESIAN_POINT('Ctrl Pts',(-20.7178168245224,18.4719590336516,
-15.6456712648569));
#104107=CARTESIAN_POINT('Ctrl Pts',(-20.7161841991896,18.4675912680562,
-15.6453908991577));
#104108=CARTESIAN_POINT('Ctrl Pts',(-20.7132689666859,18.4598700189149,
-15.6448931238288));
#104109=CARTESIAN_POINT('Ctrl Pts',(-20.7119922426294,18.4565143613628,
-15.644676067746));
#104110=CARTESIAN_POINT('Ctrl Pts',(-20.7092701406456,18.4494141666352,
-15.6442152476536));
#104111=CARTESIAN_POINT('Ctrl Pts',(-20.7078226709235,18.4456705459495,
-15.6439713646552));
#104112=CARTESIAN_POINT('Ctrl Pts',(-20.7038921035767,18.4355901593818,
-15.6433122460093));
#104113=CARTESIAN_POINT('Ctrl Pts',(-20.701389104223,18.4292612774484,-15.6428958412505));
#104114=CARTESIAN_POINT('Ctrl Pts',(-20.6888792566542,18.3980705169074,
-15.6408312811603));
#104115=CARTESIAN_POINT('Ctrl Pts',(-20.6784319270672,18.3733893636911,
-15.639158653442));
#104116=CARTESIAN_POINT('Ctrl Pts',(-20.6469617702776,18.3028068447989,
-15.6342757929205));
#104117=CARTESIAN_POINT('Ctrl Pts',(-20.6247626518491,18.2574521743443,
-15.6310149539161));
#104118=CARTESIAN_POINT('Ctrl Pts',(-20.5384183036578,18.0959373215245,
-15.6190524213131));
#104119=CARTESIAN_POINT('Ctrl Pts',(-20.4650106812556,17.9850737743559,
-15.6101842164035));
#104120=CARTESIAN_POINT('Ctrl Pts',(-20.3168836929744,17.8014515478031,
-15.5948582914854));
#104121=CARTESIAN_POINT('Ctrl Pts',(-20.2462642085409,17.7259376877789,
-15.588317349334));
#104122=CARTESIAN_POINT('Ctrl Pts',(-20.1600892183973,17.6463416523253,
-15.5811566985589));
#104123=CARTESIAN_POINT('Ctrl Pts',(-20.1496786642714,17.6369160955586,
-15.5803038902374));
#104124=CARTESIAN_POINT('Ctrl Pts',(-20.1329049473999,17.6220304532301,
-15.5789489976508));
#104125=CARTESIAN_POINT('Ctrl Pts',(-20.126601939419,17.6165034920371,-15.5784441126503));
#104126=CARTESIAN_POINT('Ctrl Pts',(-20.1153950599303,17.6067935828766,
-15.577553811901));
#104127=CARTESIAN_POINT('Ctrl Pts',(-20.1105046335844,17.6025953446085,
-15.5771677634495));
#104128=CARTESIAN_POINT('Ctrl Pts',(-20.100317799796,17.5939308402806,-15.5763686612151));
#104129=CARTESIAN_POINT('Ctrl Pts',(-20.0950184815007,17.589468103267,-15.5759557553197));
#104130=CARTESIAN_POINT('Ctrl Pts',(-20.0812910591526,17.5780224765368,
-15.5748932788432));
#104131=CARTESIAN_POINT('Ctrl Pts',(-20.0728304717354,17.5710787320826,
-15.574245306069));
#104132=CARTESIAN_POINT('Ctrl Pts',(-20.0366931601273,17.5418863115454,
-15.571506101957));
#104133=CARTESIAN_POINT('Ctrl Pts',(-20.0085118658596,17.5202694787388,
-15.5694402091633));
#104134=CARTESIAN_POINT('Ctrl Pts',(-19.9330683079436,17.4653583460582,
-15.5640774022604));
#104135=CARTESIAN_POINT('Ctrl Pts',(-19.8849623675776,17.4332722515722,
-15.5608244187097));
#104136=CARTESIAN_POINT('Ctrl Pts',(-19.6972064712897,17.3188617762681,
-15.5486249040022));
#104137=CARTESIAN_POINT('Ctrl Pts',(-19.5495977439552,17.2507069971801,
-15.5400738720789));
#104138=CARTESIAN_POINT('Ctrl Pts',(-19.3750770759619,17.1932836901734,
-15.5298129570923));
#104139=CARTESIAN_POINT('Ctrl Pts',(-19.354383064877,17.1868251740805,-15.5285932223095));
#104140=CARTESIAN_POINT('Ctrl Pts',(-19.2933187371631,17.1687916054464,
-15.5249755503349));
#104141=CARTESIAN_POINT('Ctrl Pts',(-19.2527013419445,17.1580993778045,
-15.5225457863281));
#104142=CARTESIAN_POINT('Ctrl Pts',(-19.2045508106125,17.1469442240961,
-15.5196093219412));
#104143=CARTESIAN_POINT('Ctrl Pts',(-19.1972968655522,17.1453039134232,
-15.5191654544914));
#104144=CARTESIAN_POINT('Ctrl Pts',(-19.1855407644069,17.1427105824222,
-15.5184434787778));
#104145=CARTESIAN_POINT('Ctrl Pts',(-19.1810438079709,17.1417339442152,
-15.5181666883292));
#104146=CARTESIAN_POINT('Ctrl Pts',(-19.1730488029286,17.1400248863221,
-15.5176734334068));
#104147=CARTESIAN_POINT('Ctrl Pts',(-19.1695520474956,17.1392866543535,
-15.5174573049624));
#104148=CARTESIAN_POINT('Ctrl Pts',(-19.1620431914255,17.1377212423538,
-15.5169923320035));
#104149=CARTESIAN_POINT('Ctrl Pts',(-19.1580306141694,17.1368968641308,
-15.5167433370069));
#104150=CARTESIAN_POINT('Ctrl Pts',(-19.1469791602293,17.1346597689485,
-15.5160561634185));
#104151=CARTESIAN_POINT('Ctrl Pts',(-19.1399355269112,17.1332712192264,
-15.5156166430582));
#104152=CARTESIAN_POINT('Ctrl Pts',(-19.1018128282342,17.1259571354745,
-15.5132299278544));
#104153=CARTESIAN_POINT('Ctrl Pts',(-19.0706127150178,17.1206934064988,
-15.5112483986433));
#104154=CARTESIAN_POINT('Ctrl Pts',(-18.877547017244,17.0925558083017,-15.4988612161596));
#104155=CARTESIAN_POINT('Ctrl Pts',(-18.7136042464353,17.0877959674838,
-15.4878509710221));
#104156=CARTESIAN_POINT('Ctrl Pts',(-18.4341371774074,17.1120783583669,
-15.4695259829435));
#104157=CARTESIAN_POINT('Ctrl Pts',(-18.3185529945875,17.1318652262092,
-15.4620692347016));
#104158=CARTESIAN_POINT('Ctrl Pts',(-18.1913415431482,17.1646825578858,
-15.4540473729411));
#104159=CARTESIAN_POINT('Ctrl Pts',(-18.1775384202955,17.1683928912456,
-15.4531792045577));
#104160=CARTESIAN_POINT('Ctrl Pts',(-18.1556307474793,17.1745203163682,
-15.4518046499447));
#104161=CARTESIAN_POINT('Ctrl Pts',(-18.1475014623248,17.1768466226335,
-15.4512953340162));
#104162=CARTESIAN_POINT('Ctrl Pts',(-18.1331892988731,17.1810351745544,
-15.4503998915104));
#104163=CARTESIAN_POINT('Ctrl Pts',(-18.1270006352785,17.1828771083103,
-15.4500131085094));
#104164=CARTESIAN_POINT('Ctrl Pts',(-18.1142184279995,17.1867452282034,
-15.4492150519824));
#104165=CARTESIAN_POINT('Ctrl Pts',(-18.1076261587662,17.1887753856502,
-15.4488039136819));
#104166=CARTESIAN_POINT('Ctrl Pts',(-18.0907312353962,17.1940688937844,
-15.4477513239841));
#104167=CARTESIAN_POINT('Ctrl Pts',(-18.0804433536745,17.1973790060356,
-15.4471114131979));
#104168=CARTESIAN_POINT('Ctrl Pts',(-18.0376199732079,17.2115201427185,
-15.4444517005992));
#104169=CARTESIAN_POINT('Ctrl Pts',(-18.0053236262562,17.2230624305338,
-15.4424554060208));
#104170=CARTESIAN_POINT('Ctrl Pts',(-17.9219258269259,17.2551734368749,
-15.4373139603988));
#104171=CARTESIAN_POINT('Ctrl Pts',(-17.8713205594662,17.2769610048102,
-15.4342081455096));
#104172=CARTESIAN_POINT('Ctrl Pts',(-17.7229737688609,17.3478130148979,
-15.4250667778362));
#104173=CARTESIAN_POINT('Ctrl Pts',(-17.6281227471287,17.402498916286,-15.4191799645209));
#104174=CARTESIAN_POINT('Ctrl Pts',(-17.5024497821501,17.4885537432272,
-15.4108875588415));
#104175=CARTESIAN_POINT('Ctrl Pts',(-17.4677286027148,17.5139161467976,
-15.4085376252849));
#104176=CARTESIAN_POINT('Ctrl Pts',(-17.3741844465812,17.5867161333536,
-15.4019757123918));
#104177=CARTESIAN_POINT('Ctrl Pts',(-17.3170972177541,17.6362681650533,
-15.3977069332045));
#104178=CARTESIAN_POINT('Ctrl Pts',(-17.2559602276638,17.6953557283412,
-15.3926678520874));
#104179=CARTESIAN_POINT('Ctrl Pts',(-17.2491784579698,17.7019989703284,
-15.3921019723114));
#104180=CARTESIAN_POINT('Ctrl Pts',(-17.239191448581,17.7119144878543,-15.3912579151437));
#104181=CARTESIAN_POINT('Ctrl Pts',(-17.2359516702604,17.7151520200969,
-15.3909824078313));
#104182=CARTESIAN_POINT('Ctrl Pts',(-17.2302041462665,17.7209329585408,
-15.3904905597153));
#104183=CARTESIAN_POINT('Ctrl Pts',(-17.2276923059737,17.723472222634,-15.3902745476699));
#104184=CARTESIAN_POINT('Ctrl Pts',(-17.2223034774305,17.7289475311138,
-15.3898088209111));
#104185=CARTESIAN_POINT('Ctrl Pts',(-17.2194286529396,17.7318855585587,
-15.3895589504298));
#104186=CARTESIAN_POINT('Ctrl Pts',(-17.2115115029251,17.7400240496662,
-15.3888669454493));
#104187=CARTESIAN_POINT('Ctrl Pts',(-17.2064873394198,17.7452419918485,
-15.3884234384197));
#104188=CARTESIAN_POINT('Ctrl Pts',(-17.1790220933158,17.7740611246418,
-15.3859753558713));
#104189=CARTESIAN_POINT('Ctrl Pts',(-17.1571024501804,17.7981505850561,
-15.3839343700123));
#104190=CARTESIAN_POINT('Ctrl Pts',(-17.0290693836037,17.94554963541,-15.3715277002518));
#104191=CARTESIAN_POINT('Ctrl Pts',(-16.9369043730513,18.0802479167928,
-15.3605726038094));
#104192=CARTESIAN_POINT('Ctrl Pts',(-16.8066265435636,18.3275051615477,
-15.3423172877665));
#104193=CARTESIAN_POINT('Ctrl Pts',(-16.7608184932714,18.4351816475996,
-15.3348771273156));
#104194=CARTESIAN_POINT('Ctrl Pts',(-16.7196357887292,18.5596705857064,
-15.3268707027267));
#104195=CARTESIAN_POINT('Ctrl Pts',(-16.7152852961941,18.5732820827928,
-15.3260027349164));
#104196=CARTESIAN_POINT('Ctrl Pts',(-16.7085806010559,18.5950156361407,
-15.3246284368454));
#104197=CARTESIAN_POINT('Ctrl Pts',(-16.7061367255544,18.6031093671289,
-15.3241191785866));
#104198=CARTESIAN_POINT('Ctrl Pts',(-16.7019120764584,18.6174097708592,
-15.3232238031621));
#104199=CARTESIAN_POINT('Ctrl Pts',(-16.7001111017637,18.6236103165708,
-15.3228370298821));
#104200=CARTESIAN_POINT('Ctrl Pts',(-16.6964447759263,18.6364520974938,
-15.3220389605593));
#104201=CARTESIAN_POINT('Ctrl Pts',(-16.6945834588316,18.6430944121029,
-15.3216277999039));
#104202=CARTESIAN_POINT('Ctrl Pts',(-16.6898890396264,18.6601677113828,
-15.3205750849723));
#104203=CARTESIAN_POINT('Ctrl Pts',(-16.6871032748519,18.6706115918716,
-15.319935072027));
#104204=CARTESIAN_POINT('Ctrl Pts',(-16.6758102279252,18.7142900780257,
-15.3172743666684));
#104205=CARTESIAN_POINT('Ctrl Pts',(-16.6680311460616,18.7477087572289,
-15.3152772038945));
#104206=CARTESIAN_POINT('Ctrl Pts',(-16.6498821954173,18.8352624750939,
-15.3101330168604));
#104207=CARTESIAN_POINT('Ctrl Pts',(-16.6408076226018,18.8896403453458,
-15.3070253837888));
#104208=CARTESIAN_POINT('Ctrl Pts',(-16.6200900076392,19.052789931724,-15.2978808439784));
#104209=CARTESIAN_POINT('Ctrl Pts',(-16.6147400481349,19.1621735582841,
-15.2919926661931));
#104210=CARTESIAN_POINT('Ctrl Pts',(-16.6191737846339,19.3173043946737,
-15.283543238948));
#104211=CARTESIAN_POINT('Ctrl Pts',(-16.6219715227188,19.3630724080842,
-15.2810366307503));
#104212=CARTESIAN_POINT('Ctrl Pts',(-16.6283562011198,19.4311374961686,
-15.2772455466786));
#104213=CARTESIAN_POINT('Ctrl Pts',(-16.6308174730751,19.4535273869175,
-15.2759881540931));
#104214=CARTESIAN_POINT('Ctrl Pts',(-16.6343130939643,19.4812466090109,
-15.2744141699683));
#104215=CARTESIAN_POINT('Ctrl Pts',(-16.635011342242,19.4866173921058,-15.2741083914689));
#104216=CARTESIAN_POINT('Ctrl Pts',(-16.641870248778,19.5378365537514,-15.2711840885424));
#104217=CARTESIAN_POINT('Ctrl Pts',(-16.6495110780611,19.5834704979407,
-15.2685159661971));
#104218=CARTESIAN_POINT('Ctrl Pts',(-16.6601495111548,19.6363136234963,
-15.2653150264971));
#104219=CARTESIAN_POINT('Ctrl Pts',(-16.6617000185425,19.6438051654805,
-15.2648585993042));
#104220=CARTESIAN_POINT('Ctrl Pts',(-16.6642510783471,19.6558029991519,
-15.2641231606477));
#104221=CARTESIAN_POINT('Ctrl Pts',(-16.6652258393206,19.6603147871134,
-15.2638455843075));
#104222=CARTESIAN_POINT('Ctrl Pts',(-16.6669836884761,19.6683241896854,
-15.2633509645767));
#104223=CARTESIAN_POINT('Ctrl Pts',(-16.6677609120144,19.6718230437841,
-15.2631342592713));
#104224=CARTESIAN_POINT('Ctrl Pts',(-16.6694332321476,19.6792620920397,
-15.262672144375));
#104225=CARTESIAN_POINT('Ctrl Pts',(-16.6703307107583,19.6832016410085,
-15.2624266054654));
#104226=CARTESIAN_POINT('Ctrl Pts',(-16.6727972955143,19.6938875508798,
-15.26175842468));
#104227=CARTESIAN_POINT('Ctrl Pts',(-16.674388225969,19.70062875016,-15.2613345590264));
#104228=CARTESIAN_POINT('Ctrl Pts',(-16.6826401178331,19.7348422796405,
-15.2591718208114));
#104229=CARTESIAN_POINT('Ctrl Pts',(-16.6898174407134,19.7621856161581,
-15.2574056543473));
#104230=CARTESIAN_POINT('Ctrl Pts',(-16.7124737584914,19.8419585274427,
-15.2521580326998));
#104231=CARTESIAN_POINT('Ctrl Pts',(-16.7294379277261,19.8939400342096,
-15.2486173147502));
#104232=CARTESIAN_POINT('Ctrl Pts',(-16.7969574938312,20.0765425478217,
-15.2358708234296));
#104233=CARTESIAN_POINT('Ctrl Pts',(-16.8584386647835,20.2027520771617,
-15.2265121793544));
#104234=CARTESIAN_POINT('Ctrl Pts',(-16.9794654213565,20.3990661126379,
-15.2116199811475));
#104235=CARTESIAN_POINT('Ctrl Pts',(-17.0319007420379,20.4730437999755,
-15.2059105313524));
#104236=CARTESIAN_POINT('Ctrl Pts',(-17.0975634218495,20.5541131212728,
-15.1995450771182));
#104237=CARTESIAN_POINT('Ctrl Pts',(-17.106309273107,20.5646988004627,-15.1987114833928));
#104238=CARTESIAN_POINT('Ctrl Pts',(-17.1205006703183,20.5815391861825,
-15.1973812319582));
#104239=CARTESIAN_POINT('Ctrl Pts',(-17.1258809419757,20.587848156486,-15.1968819311436));
#104240=CARTESIAN_POINT('Ctrl Pts',(-17.1354999104626,20.5989941724697,
-15.1959980725814));
#104241=CARTESIAN_POINT('Ctrl Pts',(-17.1397238194306,20.6038437889962,
-15.19561291189));
#104242=CARTESIAN_POINT('Ctrl Pts',(-17.1485707201346,20.6139082518532,
-15.1948123003579));
#104243=CARTESIAN_POINT('Ctrl Pts',(-17.1531975003402,20.6191196765284,
-15.1943970140317));
#104244=CARTESIAN_POINT('Ctrl Pts',(-17.165280276463,20.6325946339432,-15.193321264405));
#104245=CARTESIAN_POINT('Ctrl Pts',(-17.1727759166771,20.6408224515919,
-15.1926624768624));
#104246=CARTESIAN_POINT('Ctrl Pts',(-17.2056123325233,20.6763002495685,
-15.1898128466431));
#104247=CARTESIAN_POINT('Ctrl Pts',(-17.2316051358671,20.7029395445369,
-15.187650012579));
#104248=CARTESIAN_POINT('Ctrl Pts',(-17.3025263697019,20.7718904824002,
-15.1819733226059));
#104249=CARTESIAN_POINT('Ctrl Pts',(-17.3486259695994,20.8129474098401,
-15.1785104452991));
#104250=CARTESIAN_POINT('Ctrl Pts',(-17.5104278068789,20.9448338876838,
-15.166961709866));
#104251=CARTESIAN_POINT('Ctrl Pts',(-17.6337607069408,21.0256016578497,
-15.1591629772735));
#104252=CARTESIAN_POINT('Ctrl Pts',(-17.8274744164432,21.1253993391489,
-15.147064796921));
#104253=CARTESIAN_POINT('Ctrl Pts',(-17.8920713264597,21.1546736852139,
-15.1430467139788));
#104254=CARTESIAN_POINT('Ctrl Pts',(-17.9667282691337,21.1840866584231,
-15.1382899589672));
#104255=CARTESIAN_POINT('Ctrl Pts',(-17.9754722938887,21.187464667627,-15.1377311162406));
#104256=CARTESIAN_POINT('Ctrl Pts',(-17.9884995634204,21.1923982088129,
-15.1368955711384));
#104257=CARTESIAN_POINT('Ctrl Pts',(-17.9927659989993,21.1939982142445,
-15.1366214612221));
#104258=CARTESIAN_POINT('Ctrl Pts',(-18.0003838887938,21.1968270679341,
-15.1361311363564));
#104259=CARTESIAN_POINT('Ctrl Pts',(-18.0037333166834,21.1980612253662,
-15.1359152422406));
#104260=CARTESIAN_POINT('Ctrl Pts',(-18.0109615227773,21.2007038444484,
-15.1354486543612));
#104261=CARTESIAN_POINT('Ctrl Pts',(-18.0148412467138,21.202109418153,-15.1351977989155));
#104262=CARTESIAN_POINT('Ctrl Pts',(-18.0256109851437,21.2059755714557,
-15.1345003473762));
#104263=CARTESIAN_POINT('Ctrl Pts',(-18.0325096063712,21.2084117630383,
-15.1340523437058));
#104264=CARTESIAN_POINT('Ctrl Pts',(-18.0712095170149,21.2218531061725,
-15.1315327162058));
#104265=CARTESIAN_POINT('Ctrl Pts',(-18.1032551577965,21.2321338617533,
-15.1294221817715));
#104266=CARTESIAN_POINT('Ctrl Pts',(-18.2042671095229,21.261904007625,-15.122723616981));
#104267=CARTESIAN_POINT('Ctrl Pts',(-18.2739839520058,21.2786576104987,
-15.118035704664));
#104268=CARTESIAN_POINT('Ctrl Pts',(-18.3777810722535,21.298091207421,-15.1110758457956));
#104269=CARTESIAN_POINT('Ctrl Pts',(-18.4112969631768,21.3035353902479,
-15.1088312050503));
#104270=CARTESIAN_POINT('Ctrl Pts',(-18.6037233048588,21.3300591482202,
-15.0959961469476));
#104271=CARTESIAN_POINT('Ctrl Pts',(-18.7645182794458,21.3338448929013,
-15.0855309903439));
#104272=CARTESIAN_POINT('Ctrl Pts',(-18.9479199692896,21.3172985122424,
-15.0741875086963));
#104273=CARTESIAN_POINT('Ctrl Pts',(-18.971581157919,21.3147610229872,-15.0727341904368));
#104274=CARTESIAN_POINT('Ctrl Pts',(-19.0048009697951,21.3106308079139,
-15.0707072975702));
#104275=CARTESIAN_POINT('Ctrl Pts',(-19.0143984375491,21.3093706574082,
-15.0701233031633));
#104276=CARTESIAN_POINT('Ctrl Pts',(-19.0299217774807,21.3072240328976,
-15.0691812189221));
#104277=CARTESIAN_POINT('Ctrl Pts',(-19.035853039956,21.3063781610729,-15.0688218511279));
#104278=CARTESIAN_POINT('Ctrl Pts',(-19.0482160149348,21.3045614640503,
-15.0680739952793));
#104279=CARTESIAN_POINT('Ctrl Pts',(-19.0546470125605,21.3035861517726,
-15.0676856534539));
#104280=CARTESIAN_POINT('Ctrl Pts',(-19.0698542357747,21.301208104374,-15.0667689114509));
#104281=CARTESIAN_POINT('Ctrl Pts',(-19.078626368772,21.2997797052096,-15.0662413303213));
#104282=CARTESIAN_POINT('Ctrl Pts',(-19.1077750250325,21.294844696358,-15.0644921567071));
#104283=CARTESIAN_POINT('Ctrl Pts',(-19.1281095506223,21.2910947561702,
-15.0632782892737));
#104284=CARTESIAN_POINT('Ctrl Pts',(-19.2361434660464,21.2695308036851,
-15.0568586383729));
#104285=CARTESIAN_POINT('Ctrl Pts',(-19.3227069606713,21.2464665043813,
-15.0518238437803));
#104286=CARTESIAN_POINT('Ctrl Pts',(-19.5301703330354,21.1768404390375,
-15.0397511342009));
#104287=CARTESIAN_POINT('Ctrl Pts',(-19.6487483414779,21.1245437973843,
-15.0328533531562));
#104288=CARTESIAN_POINT('Ctrl Pts',(-19.8334989142043,21.0219432352675,
-15.0211964060819));
#104289=CARTESIAN_POINT('Ctrl Pts',(-19.9028057015225,20.9780040494487,
-15.0165828658396));
#104290=CARTESIAN_POINT('Ctrl Pts',(-19.9771545516593,20.9245773642244,
-15.0111575673033));
#104291=CARTESIAN_POINT('Ctrl Pts',(-19.9848895678032,20.918939080845,-15.0105870717844));
#104292=CARTESIAN_POINT('Ctrl Pts',(-19.9962811381506,20.9105165334373,
-15.0097374358223));
#104293=CARTESIAN_POINT('Ctrl Pts',(-19.9999674132718,20.9077724145501,
-15.0094610169595));
#104294=CARTESIAN_POINT('Ctrl Pts',(-20.0063837373337,20.902963457562,-15.0089772389423));
#104295=CARTESIAN_POINT('Ctrl Pts',(-20.0091177490575,20.9009039743805,
-15.008770255574));
#104296=CARTESIAN_POINT('Ctrl Pts',(-20.0150075412379,20.8964448658886,
-15.0083225160251));
#104297=CARTESIAN_POINT('Ctrl Pts',(-20.0181615319694,20.8940430404099,
-15.0080816086366));
#104298=CARTESIAN_POINT('Ctrl Pts',(-20.0265244494044,20.8876373227478,
-15.0074398345719));
#104299=CARTESIAN_POINT('Ctrl Pts',(-20.0317214665898,20.8836180546893,
-15.0070379060703));
#104300=CARTESIAN_POINT('Ctrl Pts',(-20.0432646057647,20.8746046426172,
-15.0061383884991));
#104301=CARTESIAN_POINT('Ctrl Pts',(-20.0496009979838,20.8695982709328,
-15.0056399955571));
#104302=CARTESIAN_POINT('Ctrl Pts',(-20.0687009852409,20.8543290951319,
-15.0041240226512));
#104303=CARTESIAN_POINT('Ctrl Pts',(-20.081373976043,20.8439545519783,-15.0030995363081));
#104304=CARTESIAN_POINT('Ctrl Pts',(-20.1281089704422,20.8047812675753,
-14.9992554749572));
#104305=CARTESIAN_POINT('Ctrl Pts',(-20.1613768482111,20.7750567053641,
-14.9963865431328));
#104306=CARTESIAN_POINT('Ctrl Pts',(-20.2445526816772,20.6958748397315,
-14.9889148943829));
#104307=CARTESIAN_POINT('Ctrl Pts',(-20.2929831227089,20.6449434280133,
-14.9842691881742));
#104308=CARTESIAN_POINT('Ctrl Pts',(-20.4440854126164,20.4693169760868,
-14.9689598573328));
#104309=CARTESIAN_POINT('Ctrl Pts',(-20.5350536727807,20.3352677094884,
-14.9584150521823));
#104310=CARTESIAN_POINT('Ctrl Pts',(-20.620913479345,20.1711097446328,-14.9470037008193));
#104311=CARTESIAN_POINT('Ctrl Pts',(-20.6315674586002,20.1498775279336,
-14.9455529591341));
#104312=CARTESIAN_POINT('Ctrl Pts',(-20.646054146623,20.1197527168517,-14.9435290278956));
#104313=CARTESIAN_POINT('Ctrl Pts',(-20.6501863570855,20.1110068942963,
-14.9429454590489));
#104314=CARTESIAN_POINT('Ctrl Pts',(-20.6567802224698,20.0967996924775,
-14.9420038768959));
#104315=CARTESIAN_POINT('Ctrl Pts',(-20.6592788587166,20.0913557215352,
-14.9416445882744));
#104316=CARTESIAN_POINT('Ctrl Pts',(-20.6644429061992,20.0799772762732,
-14.940896753786));
#104317=CARTESIAN_POINT('Ctrl Pts',(-20.6671041392669,20.074040965992,-14.9405083547772));
#104318=CARTESIAN_POINT('Ctrl Pts',(-20.6733384837056,20.0599607373865,
-14.9395912218884));
#104319=CARTESIAN_POINT('Ctrl Pts',(-20.6768877434239,20.0518063440148,
-14.9390633090039));
#104320=CARTESIAN_POINT('Ctrl Pts',(-20.6885303668951,20.0245901237712,
-14.9373118791438));
#104321=CARTESIAN_POINT('Ctrl Pts',(-20.6963955738974,20.005431558431,-14.936096115036));
#104322=CARTESIAN_POINT('Ctrl Pts',(-20.7368428455887,19.9026395615762,
-14.9296592930422));
#104323=CARTESIAN_POINT('Ctrl Pts',(-20.7643644939504,19.8171084338586,
-14.9246102958648));
#104324=CARTESIAN_POINT('Ctrl Pts',(-20.8293843562145,19.5600283275059,
-14.9099831155574));
#104325=CARTESIAN_POINT('Ctrl Pts',(-20.8510852885873,19.3853205293609,
-14.9007777448692));
#104326=CARTESIAN_POINT('Ctrl Pts',(-20.8509997481126,19.2099672893213,
-14.890777245922));
#104327=CARTESIAN_POINT('Ctrl Pts',(-20.8509997467292,19.2099644573727,
-14.8907770844143));
#104328=CARTESIAN_POINT('Ctrl Pts',(-20.8509866388053,19.1831674228977,
-14.8892488323634));
#104329=CARTESIAN_POINT('Ctrl Pts',(-20.8504647358832,19.1563740229349,
-14.8877018835943));
#104330=CARTESIAN_POINT('Ctrl Pts',(-20.8488772352135,19.1151184590359,
-14.8852810654424));
#104331=CARTESIAN_POINT('Ctrl Pts',(-20.848171390759,19.1006446878675,-14.8844243778208));
#104332=CARTESIAN_POINT('Ctrl Pts',(-20.8470399811955,19.0814889254113,
-14.8832794438788));
#104333=CARTESIAN_POINT('Ctrl Pts',(-20.846747309812,19.0767990890141,-14.8829982498832));
#104334=CARTESIAN_POINT('Ctrl Pts',(-20.8462061822037,19.0685688227447,
-14.8825031657956));
#104335=CARTESIAN_POINT('Ctrl Pts',(-20.845964430718,19.0650279500911,-14.8822896436915));
#104336=CARTESIAN_POINT('Ctrl Pts',(-20.8454718256797,19.0580703882878,
-14.8818690285064));
#104337=CARTESIAN_POINT('Ctrl Pts',(-20.8452215797105,19.054653660018,-14.8816619690076));
#104338=CARTESIAN_POINT('Ctrl Pts',(-20.8446669325024,19.0473250308869,
-14.8812167390628));
#104339=CARTESIAN_POINT('Ctrl Pts',(-20.8443599503408,19.0434133809311,
-14.8809784276841));
#104340=CARTESIAN_POINT('Ctrl Pts',(-20.8435234722957,19.0331216543962,
-14.8803496960766));
#104341=CARTESIAN_POINT('Ctrl Pts',(-20.842975911369,19.0267431444018,-14.8799582825531));
#104342=CARTESIAN_POINT('Ctrl Pts',(-20.840583202641,19.0002797620154,-14.8783274067943));
#104343=CARTESIAN_POINT('Ctrl Pts',(-20.8384800650701,18.980220028178,-14.8770745123902));
#104344=CARTESIAN_POINT('Ctrl Pts',(-20.8355857356411,18.9559616381952,
-14.8755416340987));
#104345=CARTESIAN_POINT('Ctrl Pts',(-20.8350679505098,18.9517305706445,
-14.87527361885));
#104346=CARTESIAN_POINT('Ctrl Pts',(-20.8313092224031,18.9217670685447,
-14.8733710788059));
#104347=CARTESIAN_POINT('Ctrl Pts',(-20.8276085450745,18.8960955537747,
-14.8717174824157));
#104348=CARTESIAN_POINT('Ctrl Pts',(-20.8020052665551,18.7389842819775,
-14.8614773236772));
#104349=CARTESIAN_POINT('Ctrl Pts',(-20.7682207967035,18.6098833818227,
-14.8525677679027));
#104350=CARTESIAN_POINT('Ctrl Pts',(-20.7225806190038,18.4848897317057,
-14.8438386123028));
#104351=CARTESIAN_POINT('Origin',(-18.734,19.211,0.));
#104352=CARTESIAN_POINT('',(-20.7225806179957,18.4848897289449,-14.042655348398));
#104353=CARTESIAN_POINT('',(-20.7225806137986,18.4848897174502,-14.2664527203653));
#104354=CARTESIAN_POINT('',(-20.7225806137986,18.4848897174502,0.));
#104355=CARTESIAN_POINT('',(-20.8484261613494,19.2114672066158,-14.3109440134323));
#104356=CARTESIAN_POINT('Ctrl Pts',(-20.7225806137986,18.4848897174502,
-14.2664527203653));
#104357=CARTESIAN_POINT('Ctrl Pts',(-20.7483493632785,18.5554619664447,
-14.2709758355722));
#104358=CARTESIAN_POINT('Ctrl Pts',(-20.7703907027832,18.6274990086842,
-14.2754989507791));
#104359=CARTESIAN_POINT('Ctrl Pts',(-20.7885479544131,18.7005867331105,
-14.280022065986));
#104360=CARTESIAN_POINT('Ctrl Pts',(-20.8066819175929,18.7735807153857,
-14.2845393798555));
#104361=CARTESIAN_POINT('Ctrl Pts',(-20.8209415894746,18.8476222797955,
-14.289056693725));
#104362=CARTESIAN_POINT('Ctrl Pts',(-20.8312196705739,18.9222810131672,
-14.2935740075945));
#104363=CARTESIAN_POINT('Ctrl Pts',(-20.8414842530404,18.9968416941083,
-14.2980853886872));
#104364=CARTESIAN_POINT('Ctrl Pts',(-20.8477775921481,19.0720174996117,
-14.3025967697798));
#104365=CARTESIAN_POINT('Ctrl Pts',(-20.8500434728548,19.1473680819993,
-14.3071081508725));
#104366=CARTESIAN_POINT('Ctrl Pts',(-20.8506856224259,19.1687224030869,
-14.3083866742408));
#104367=CARTESIAN_POINT('Ctrl Pts',(-20.8510046224853,19.1900907116534,
-14.3096651976092));
#104368=CARTESIAN_POINT('Ctrl Pts',(-20.850999949394,19.2114628884564,-14.3109437209775));
#104369=CARTESIAN_POINT('Ctrl Pts',(-20.8476071148151,19.2114685807669,
-14.310944106499));
#104370=CARTESIAN_POINT('Ctrl Pts',(-20.8482399645881,19.5369557946072,
-14.3304466040373));
#104371=CARTESIAN_POINT('Ctrl Pts',(-20.6243347143573,20.5691167586125,
-14.3923410371361));
#104372=CARTESIAN_POINT('Ctrl Pts',(-19.0148744787981,21.6984565315257,
-14.4966274057954));
#104373=CARTESIAN_POINT('Ctrl Pts',(-16.7944747336858,20.7935840294886,
-14.6238032124768));
#104374=CARTESIAN_POINT('Ctrl Pts',(-16.3534690399024,18.4367889066407,
-14.7509790191583));
#104375=CARTESIAN_POINT('Ctrl Pts',(-18.0964527495932,16.7902844089888,
-14.8781548258396));
#104376=CARTESIAN_POINT('Ctrl Pts',(-20.0208839008303,17.2650915259889,
-14.9832889561996));
#104377=CARTESIAN_POINT('Ctrl Pts',(-20.6031710249408,18.1668852825214,
-15.0460311509992));
#104378=CARTESIAN_POINT('Ctrl Pts',(-20.7193263794245,18.4860708438863,
-15.0663814102382));
#104379=CARTESIAN_POINT('Ctrl Pts',(-20.7225806190038,18.4848897317057,
-14.8438386123028));
#104380=CARTESIAN_POINT('Ctrl Pts',(-20.7074810939562,18.4435370278851,
-14.8409506721092));
#104381=CARTESIAN_POINT('Ctrl Pts',(-20.6910839087439,18.4026340477406,
-14.8380800866817));
#104382=CARTESIAN_POINT('Ctrl Pts',(-20.6498725442178,18.3084662526309,
-14.8314542563252));
#104383=CARTESIAN_POINT('Ctrl Pts',(-20.6241100173458,18.2556885989155,
-14.8277280609254));
#104384=CARTESIAN_POINT('Ctrl Pts',(-20.5791049394694,18.1724595813546,
-14.8218389175388));
#104385=CARTESIAN_POINT('Ctrl Pts',(-20.5612232428029,18.1413113033745,
-14.8196315672646));
#104386=CARTESIAN_POINT('Ctrl Pts',(-20.5368450703277,18.1012435357112,
-14.816785900081));
#104387=CARTESIAN_POINT('Ctrl Pts',(-20.5310601569201,18.0919001129576,
-14.8161218507982));
#104388=CARTESIAN_POINT('Ctrl Pts',(-20.5215047349287,18.0767319740383,
-14.8150429449288));
#104389=CARTESIAN_POINT('Ctrl Pts',(-20.5177779362274,18.0708800904631,
-14.8146264839918));
#104390=CARTESIAN_POINT('Ctrl Pts',(-20.5105354664624,18.0596302803133,
-14.8138254046825));
#104391=CARTESIAN_POINT('Ctrl Pts',(-20.5070237974983,18.0542298802567,
-14.8134406434552));
#104392=CARTESIAN_POINT('Ctrl Pts',(-20.4988979148387,18.0418574733217,
-14.8125586240517));
#104393=CARTESIAN_POINT('Ctrl Pts',(-20.494266920987,18.0348965745188,-14.8120620011086));
#104394=CARTESIAN_POINT('Ctrl Pts',(-20.481790053944,18.0163812394956,-14.8107398688276));
#104395=CARTESIAN_POINT('Ctrl Pts',(-20.4738707904637,18.0048765809252,
-14.8099171340184));
#104396=CARTESIAN_POINT('Ctrl Pts',(-20.4096460920631,17.9135235647273,
-14.8033723417588));
#104397=CARTESIAN_POINT('Ctrl Pts',(-20.3479848091841,17.8375767418352,
-14.7978661273312));
#104398=CARTESIAN_POINT('Ctrl Pts',(-20.1877542516837,17.665985351725,-14.7849162800294));
#104399=CARTESIAN_POINT('Ctrl Pts',(-20.0847171457458,17.5751416781252,
-14.7776254632276));
#104400=CARTESIAN_POINT('Ctrl Pts',(-19.9319513590194,17.4647913235688,
-14.7671839048302));
#104401=CARTESIAN_POINT('Ctrl Pts',(-19.8891950784322,17.4362166838002,
-14.7642935827439));
#104402=CARTESIAN_POINT('Ctrl Pts',(-19.8301035963785,17.3997653948343,
-14.7602823390455));
#104403=CARTESIAN_POINT('Ctrl Pts',(-19.8146431415058,17.390498902606,-14.7592313479842));
#104404=CARTESIAN_POINT('Ctrl Pts',(-19.7915920186869,17.3770799012701,
-14.757659271722));
#104405=CARTESIAN_POINT('Ctrl Pts',(-19.7840907938231,17.3727744627639,
-14.7571469071607));
#104406=CARTESIAN_POINT('Ctrl Pts',(-19.7704624556153,17.3650629156234,
-14.7562142311961));
#104407=CARTESIAN_POINT('Ctrl Pts',(-19.764344362987,17.3616410213517,-14.7557948778035));
#104408=CARTESIAN_POINT('Ctrl Pts',(-19.7546790594241,17.3562979941646,
-14.7551311818541));
#104409=CARTESIAN_POINT('Ctrl Pts',(-19.7511430959116,17.3543564707753,
-14.754888122013));
#104410=CARTESIAN_POINT('Ctrl Pts',(-19.7475925566865,17.3524201310848,
-14.7546437854131));
#104411=CARTESIAN_POINT('Ctrl Pts',(-19.7475834744231,17.352415178023,-14.7546431603994));
#104412=CARTESIAN_POINT('Ctrl Pts',(-19.7475652544736,17.3524052418474,
-14.7546419065543));
#104413=CARTESIAN_POINT('Ctrl Pts',(-19.7475561170615,17.3524002588843,
-14.7546412777418));
#104414=CARTESIAN_POINT('Ctrl Pts',(-19.7475377863691,17.3523902626663,
-14.7546400162684));
#104415=CARTESIAN_POINT('Ctrl Pts',(-19.747528593265,17.3523852495087,-14.7546393836196));
#104416=CARTESIAN_POINT('Ctrl Pts',(-19.7475101508872,17.3523751927407,
-14.7546381144528));
#104417=CARTESIAN_POINT('Ctrl Pts',(-19.747500901695,17.3523701491759,-14.7546374779405));
#104418=CARTESIAN_POINT('Ctrl Pts',(-19.7474823468813,17.3523600314552,
-14.7546362010287));
#104419=CARTESIAN_POINT('Ctrl Pts',(-19.7474730411775,17.3523549572555,
-14.7546355606235));
#104420=CARTESIAN_POINT('Ctrl Pts',(-19.7474543727597,17.3523447779515,
-14.754634275886));
#104421=CARTESIAN_POINT('Ctrl Pts',(-19.7474450103116,17.3523396729934,
-14.754633631572));
#104422=CARTESIAN_POINT('Ctrl Pts',(-19.7474262281966,17.3523294320622,
-14.7546323390023));
#104423=CARTESIAN_POINT('Ctrl Pts',(-19.7474168083247,17.3523242959784,
-14.7546316907326));
#104424=CARTESIAN_POINT('Ctrl Pts',(-19.7473979109353,17.3523139925667,
-14.7546303902221));
#104425=CARTESIAN_POINT('Ctrl Pts',(-19.7473884334741,17.3523088252705,
-14.7546297379852));
#104426=CARTESIAN_POINT('Ctrl Pts',(-19.7473694205619,17.3522984592496,
-14.7546284295165));
#104427=CARTESIAN_POINT('Ctrl Pts',(-19.7473598849335,17.3522932604293,
-14.7546277732726));
#104428=CARTESIAN_POINT('Ctrl Pts',(-19.7473407551873,17.3522828310914,
-14.7546264567555));
#104429=CARTESIAN_POINT('Ctrl Pts',(-19.7473311611348,17.3522776006104,
-14.7546257964868));
#104430=CARTESIAN_POINT('Ctrl Pts',(-19.7473119141314,17.3522671077316,
-14.7546244718919));
#104431=CARTESIAN_POINT('Ctrl Pts',(-19.7473022611091,17.3522618452961,
-14.7546238075608));
#104432=CARTESIAN_POINT('Ctrl Pts',(-19.747282895701,17.3522512882581,-14.754622474809));
#104433=CARTESIAN_POINT('Ctrl Pts',(-19.7472731833765,17.3522459936903,
-14.7546218063925));
#104434=CARTESIAN_POINT('Ctrl Pts',(-19.7472537367182,17.3522353927542,
-14.7546204680408));
#104435=CARTESIAN_POINT('Ctrl Pts',(-19.7472439456494,17.3522300554586,
-14.7546197942006));
#104436=CARTESIAN_POINT('Ctrl Pts',(-19.7472243210675,17.3522193579327,
-14.7546184435955));
#104437=CARTESIAN_POINT('Ctrl Pts',(-19.7472144893949,17.3522139987059,
-14.7546177669569));
#104438=CARTESIAN_POINT('Ctrl Pts',(-19.7471947638124,17.3522032465298,
-14.7546164093922));
#104439=CARTESIAN_POINT('Ctrl Pts',(-19.7471848713441,17.3521978543676,
-14.7546157285652));
#104440=CARTESIAN_POINT('Ctrl Pts',(-19.7471650238516,17.3521870361508,
-14.7546143626018));
#104441=CARTESIAN_POINT('Ctrl Pts',(-19.7471550703389,17.3521816109215,
-14.7546136775693));
#104442=CARTESIAN_POINT('Ctrl Pts',(-19.7471350678491,17.3521707086376,
-14.7546123009297));
#104443=CARTESIAN_POINT('Ctrl Pts',(-19.7471250690313,17.3521652589243,
-14.754611612775));
#104444=CARTESIAN_POINT('Ctrl Pts',(-19.7441124399662,17.3505232996412,
-14.7544042720479));
#104445=CARTESIAN_POINT('Ctrl Pts',(-19.7411059130456,17.3488941025673,
-14.7541971504298));
#104446=CARTESIAN_POINT('Ctrl Pts',(-19.7340553278126,17.345095553937,-14.7537109715613));
#104447=CARTESIAN_POINT('Ctrl Pts',(-19.7300081664629,17.3429320697717,
-14.7534315464017));
#104448=CARTESIAN_POINT('Ctrl Pts',(-19.7175267213398,17.3363119759748,
-14.7525687997221));
#104449=CARTESIAN_POINT('Ctrl Pts',(-19.7090694601547,17.3318992738382,
-14.7519828138157));
#104450=CARTESIAN_POINT('Ctrl Pts',(-19.5956003752683,17.2736673480883,
-14.7441050453644));
#104451=CARTESIAN_POINT('Ctrl Pts',(-19.4863089443862,17.2286686009833,
-14.7363487722729));
#104452=CARTESIAN_POINT('Ctrl Pts',(-19.2694538392336,17.1599092270964,
-14.721321551487));
#104453=CARTESIAN_POINT('Ctrl Pts',(-19.1626341486267,17.1349555878662,
-14.7140786555689));
#104454=CARTESIAN_POINT('Ctrl Pts',(-18.9793306433264,17.1068938237246,
-14.7021574895197));
#104455=CARTESIAN_POINT('Ctrl Pts',(-18.9037343106975,17.0994502355644,
-14.6973801126354));
#104456=CARTESIAN_POINT('Ctrl Pts',(-18.8089876374995,17.0952438713994,
-14.6915694461902));
#104457=CARTESIAN_POINT('Ctrl Pts',(-18.7900707676563,17.0946580505478,
-14.6904178947741));
#104458=CARTESIAN_POINT('Ctrl Pts',(-18.7625736042103,17.0941754693399,
-14.6887560549823));
#104459=CARTESIAN_POINT('Ctrl Pts',(-18.7539981860228,17.0940770868078,
-14.6882394819095));
#104460=CARTESIAN_POINT('Ctrl Pts',(-18.7389698607122,17.0939960000606,
-14.6873371006462));
#104461=CARTESIAN_POINT('Ctrl Pts',(-18.7325172344247,17.0939906853981,
-14.6869505893649));
#104462=CARTESIAN_POINT('Ctrl Pts',(-18.7199933870443,17.0940376301673,
-14.6862021993523));
#104463=CARTESIAN_POINT('Ctrl Pts',(-18.7139222233543,17.0940865051778,
-14.6858402184515));
#104464=CARTESIAN_POINT('Ctrl Pts',(-18.6994183944424,17.0942656667909,
-14.6849773628794));
#104465=CARTESIAN_POINT('Ctrl Pts',(-18.6909860909016,17.0944202279193,
-14.6844772515407));
#104466=CARTESIAN_POINT('Ctrl Pts',(-18.6606154304775,17.0951584825035,
-14.6826813631511));
#104467=CARTESIAN_POINT('Ctrl Pts',(-18.6386850642242,17.09603292263,-14.68139467265));
#104468=CARTESIAN_POINT('Ctrl Pts',(-18.4298946557656,17.1076124082181,
-14.6692307348517));
#104469=CARTESIAN_POINT('Ctrl Pts',(-18.245223051317,17.1427102761129,-14.6592274597903));
#104470=CARTESIAN_POINT('Ctrl Pts',(-17.9924737538082,17.2265388712724,
-14.6447059452045));
#104471=CARTESIAN_POINT('Ctrl Pts',(-17.9188479796461,17.2556298614884,
-14.6403524532702));
#104472=CARTESIAN_POINT('Ctrl Pts',(-17.8145678378771,17.3037476375967,
-14.6337811992519));
#104473=CARTESIAN_POINT('Ctrl Pts',(-17.7824935359329,17.3195449562838,
-14.6317013004945));
#104474=CARTESIAN_POINT('Ctrl Pts',(-17.7442395922749,17.3396051122237,
-14.6291306492335));
#104475=CARTESIAN_POINT('Ctrl Pts',(-17.7376608529344,17.3430993626594,
-14.6286852813754));
#104476=CARTESIAN_POINT('Ctrl Pts',(-17.7274410974989,17.3485968629561,
-14.6279880876208));
#104477=CARTESIAN_POINT('Ctrl Pts',(-17.7237872320985,17.350576276231,-14.6277377511103));
#104478=CARTESIAN_POINT('Ctrl Pts',(-17.7170085455672,17.3542743605943,
-14.6272712903984));
#104479=CARTESIAN_POINT('Ctrl Pts',(-17.7138822307273,17.3559901739827,
-14.6270553484315));
#104480=CARTESIAN_POINT('Ctrl Pts',(-17.7068071634323,17.3598964731108,
-14.6265648215043));
#104481=CARTESIAN_POINT('Ctrl Pts',(-17.7028610945467,17.3620916876317,
-14.6262899372727));
#104482=CARTESIAN_POINT('Ctrl Pts',(-17.6926827798906,17.3677966453459,
-14.6255776181735));
#104483=CARTESIAN_POINT('Ctrl Pts',(-17.686461302725,17.371325345643,-14.6251390092721));
#104484=CARTESIAN_POINT('Ctrl Pts',(-17.6481989292703,17.3932840369426,
-14.622422289333));
#104485=CARTESIAN_POINT('Ctrl Pts',(-17.6166294671786,17.4125178627682,
-14.6200972369997));
#104486=CARTESIAN_POINT('Ctrl Pts',(-17.4423708657676,17.5250448420197,
-14.6068559426971));
#104487=CARTESIAN_POINT('Ctrl Pts',(-17.3108550832063,17.6344809421486,
-14.5953532433733));
#104488=CARTESIAN_POINT('Ctrl Pts',(-17.1286102227943,17.8277199462038,
-14.578093569771));
#104489=CARTESIAN_POINT('Ctrl Pts',(-17.0680690264989,17.9012602334922,
-14.5720497573367));
#104490=CARTESIAN_POINT('Ctrl Pts',(-17.0002387241461,17.9960032205012,
-14.5648925934082));
#104491=CARTESIAN_POINT('Ctrl Pts',(-16.988066558422,18.0135603122002,-14.5635905223771));
#104492=CARTESIAN_POINT('Ctrl Pts',(-16.9711439254845,18.0387762385067,
-14.5617539624484));
#104493=CARTESIAN_POINT('Ctrl Pts',(-16.9661736864758,18.0462853501422,
-14.5612111909313));
#104494=CARTESIAN_POINT('Ctrl Pts',(-16.9576845789646,18.059290355027,-14.5602782050805));
#104495=CARTESIAN_POINT('Ctrl Pts',(-16.9541429611953,18.0647711815569,
-14.5598871415699));
#104496=CARTESIAN_POINT('Ctrl Pts',(-16.9474121127944,18.0752939150927,
-14.5591403680547));
#104497=CARTESIAN_POINT('Ctrl Pts',(-16.9442187474406,18.0803330909973,
-14.5587845066282));
#104498=CARTESIAN_POINT('Ctrl Pts',(-16.9359741214643,18.0934656798873,
-14.5578616095128));
#104499=CARTESIAN_POINT('Ctrl Pts',(-16.9309561569804,18.1015799167171,
-14.5572958075361));
#104500=CARTESIAN_POINT('Ctrl Pts',(-16.9140516762329,18.1293327463225,
-14.555375388746));
#104501=CARTESIAN_POINT('Ctrl Pts',(-16.9024295377536,18.1491310573651,
-14.5540304273604));
#104502=CARTESIAN_POINT('Ctrl Pts',(-16.8045313749223,18.3222916902474,
-14.5424711530142));
#104503=CARTESIAN_POINT('Ctrl Pts',(-16.7373660541129,18.4856647684759,
-14.5330125310625));
#104504=CARTESIAN_POINT('Ctrl Pts',(-16.6684448818761,18.7391079634928,
-14.5187205459973));
#104505=CARTESIAN_POINT('Ctrl Pts',(-16.6508614700646,18.8240484142426,
-14.5139749289586));
#104506=CARTESIAN_POINT('Ctrl Pts',(-16.633164796856,18.9471732202117,-14.5068723156672));
#104507=CARTESIAN_POINT('Ctrl Pts',(-16.628796097937,18.984661195206,-14.5046801066245));
#104508=CARTESIAN_POINT('Ctrl Pts',(-16.6247571231889,19.029779848697,-14.5019849044099));
#104509=CARTESIAN_POINT('Ctrl Pts',(-16.6241228721184,19.0373199552581,
-14.5015325916766));
#104510=CARTESIAN_POINT('Ctrl Pts',(-16.6232009377204,19.0490314809562,
-14.5008268768696));
#104511=CARTESIAN_POINT('Ctrl Pts',(-16.6228851602042,19.0532007129879,
-14.5005750237261));
#104512=CARTESIAN_POINT('Ctrl Pts',(-16.6223231110824,19.0609252918407,
-14.5001072020833));
#104513=CARTESIAN_POINT('Ctrl Pts',(-16.6220734651768,19.0644803352983,
-14.4998914250786));
#104514=CARTESIAN_POINT('Ctrl Pts',(-16.6215301551055,19.0725072628519,
-14.4994031572928));
#104515=CARTESIAN_POINT('Ctrl Pts',(-16.6212417150351,19.076979433336,-14.4991303789823));
#104516=CARTESIAN_POINT('Ctrl Pts',(-16.6204343472392,19.0901482987605,
-14.4983250329178));
#104517=CARTESIAN_POINT('Ctrl Pts',(-16.6199549094181,19.0988471970192,
-14.4977903330675));
#104518=CARTESIAN_POINT('Ctrl Pts',(-16.6169286455891,19.1607018320226,
-14.4939701668306));
#104519=CARTESIAN_POINT('Ctrl Pts',(-16.6163334980486,19.2139295643992,
-14.4905880962561));
#104520=CARTESIAN_POINT('Ctrl Pts',(-16.6182286927023,19.2853989561472,
-14.485967869652));
#104521=CARTESIAN_POINT('Ctrl Pts',(-16.6189503069181,19.3036725319898,
-14.4847795540402));
#104522=CARTESIAN_POINT('Ctrl Pts',(-16.6224232250216,19.3698565795093,
-14.4804550299526));
#104523=CARTESIAN_POINT('Ctrl Pts',(-16.626566576587,19.4176785584734,-14.4772914046414));
#104524=CARTESIAN_POINT('Ctrl Pts',(-16.6454707351015,19.5739019566192,
-14.4668964299862));
#104525=CARTESIAN_POINT('Ctrl Pts',(-16.667006818079,19.6813136955979,-14.4596640531949));
#104526=CARTESIAN_POINT('Ctrl Pts',(-16.7117288233571,19.8396045538036,
-14.449091291971));
#104527=CARTESIAN_POINT('Ctrl Pts',(-16.7287731956925,19.8920217918751,
-14.4456025274249));
#104528=CARTESIAN_POINT('Ctrl Pts',(-16.7597164155145,19.975898593138,-14.4400454813959));
#104529=CARTESIAN_POINT('Ctrl Pts',(-16.7723690934829,20.0077872568148,
-14.4379387701988));
#104530=CARTESIAN_POINT('Ctrl Pts',(-16.7900208109303,20.0493022893744,
-14.435202409783));
#104531=CARTESIAN_POINT('Ctrl Pts',(-16.7943260709846,20.0592162883305,
-14.4345494228329));
#104532=CARTESIAN_POINT('Ctrl Pts',(-16.8015031187555,20.0754029070089,
-14.4334839443931));
#104533=CARTESIAN_POINT('Ctrl Pts',(-16.8043299359631,20.0816951403201,
-14.4330699235782));
#104534=CARTESIAN_POINT('Ctrl Pts',(-16.809862216762,20.0938502029877,-14.432270410746));
#104535=CARTESIAN_POINT('Ctrl Pts',(-16.8125638443236,20.0997146847468,
-14.431884792412));
#104536=CARTESIAN_POINT('Ctrl Pts',(-16.8188649676653,20.1132296223118,
-14.430996361538));
#104537=CARTESIAN_POINT('Ctrl Pts',(-16.8224835642167,20.1208710910598,
-14.4304942151134));
#104538=CARTESIAN_POINT('Ctrl Pts',(-16.8323411847198,20.1413692616423,
-14.4291475654056));
#104539=CARTESIAN_POINT('Ctrl Pts',(-16.8386648370025,20.1541849487556,
-14.4283060038041));
#104540=CARTESIAN_POINT('Ctrl Pts',(-16.8978932610095,20.2712173931745,
-14.4206218509398));
#104541=CARTESIAN_POINT('Ctrl Pts',(-16.9592165448794,20.3709559613255,
-14.4140961722568));
#104542=CARTESIAN_POINT('Ctrl Pts',(-17.1249750309179,20.5963756919772,
-14.3987786755774));
#104543=CARTESIAN_POINT('Ctrl Pts',(-17.2362957730824,20.7160240140932,
-14.3901704072727));
#104544=CARTESIAN_POINT('Ctrl Pts',(-17.3848033511061,20.8426868177589,
-14.3789607229529));
#104545=CARTESIAN_POINT('Ctrl Pts',(-17.4098681336797,20.8630920108258,
-14.3770754920012));
#104546=CARTESIAN_POINT('Ctrl Pts',(-17.4410957648968,20.8873471783227,
-14.374721124771));
#104547=CARTESIAN_POINT('Ctrl Pts',(-17.4468255676913,20.891750784859,-14.3742889082093));
#104548=CARTESIAN_POINT('Ctrl Pts',(-17.4558467345305,20.8986107655607,
-14.3736078649816));
#104549=CARTESIAN_POINT('Ctrl Pts',(-17.4591229535437,20.9010870929708,
-14.3733604177488));
#104550=CARTESIAN_POINT('Ctrl Pts',(-17.4652624476059,20.9056996149459,
-14.3728964590385));
#104551=CARTESIAN_POINT('Ctrl Pts',(-17.4681239311548,20.9078381005326,
-14.3726801118633));
#104552=CARTESIAN_POINT('Ctrl Pts',(-17.4746711169923,20.9127052607457,
-14.3721848680646));
#104553=CARTESIAN_POINT('Ctrl Pts',(-17.4783602689436,20.9154291991472,
-14.3719056480819));
#104554=CARTESIAN_POINT('Ctrl Pts',(-17.4897370124984,20.9237723998262,
-14.3710441503994));
#104555=CARTESIAN_POINT('Ctrl Pts',(-17.497453566851,20.9293517063032,-14.3704592192566));
#104556=CARTESIAN_POINT('Ctrl Pts',(-17.6027126014085,21.004381077153,-14.3624752158412));
#104557=CARTESIAN_POINT('Ctrl Pts',(-17.7059278904727,21.0654778131456,
-14.3545981896885));
#104558=CARTESIAN_POINT('Ctrl Pts',(-17.9118352095968,21.1648677277371,
-14.3394934700293));
#104559=CARTESIAN_POINT('Ctrl Pts',(-18.0134478427727,21.2045802231746,
-14.3322936454142));
#104560=CARTESIAN_POINT('Ctrl Pts',(-18.1893948081644,21.2581235480728,
-14.3204773940205));
#104561=CARTESIAN_POINT('Ctrl Pts',(-18.2622328660778,21.2761265211801,
-14.315760705147));
#104562=CARTESIAN_POINT('Ctrl Pts',(-18.3543438138816,21.2937634493328,
-14.3100154945869));
#104563=CARTESIAN_POINT('Ctrl Pts',(-18.3728541999036,21.2970527683627,
-14.3088716863477));
#104564=CARTESIAN_POINT('Ctrl Pts',(-18.3998464503934,21.3014792644285,
-14.3072189012943));
#104565=CARTESIAN_POINT('Ctrl Pts',(-18.4082948797795,21.3028122113937,
-14.3067037355036));
#104566=CARTESIAN_POINT('Ctrl Pts',(-18.4231273933581,21.3050603648378,
-14.3058029785259));
#104567=CARTESIAN_POINT('Ctrl Pts',(-18.4295079701632,21.3059976597453,
-14.3054166919703));
#104568=CARTESIAN_POINT('Ctrl Pts',(-18.4419102531478,21.307761675116,-14.3046681319736));
#104569=CARTESIAN_POINT('Ctrl Pts',(-18.4479314263017,21.3085916463361,
-14.3043057592092));
#104570=CARTESIAN_POINT('Ctrl Pts',(-18.4623409382361,21.3105146846798,
-14.3034410071946));
#104571=CARTESIAN_POINT('Ctrl Pts',(-18.4707324596797,21.3115834338094,
-14.3029393990358));
#104572=CARTESIAN_POINT('Ctrl Pts',(-18.5010776134917,21.3152635131433,
-14.301132495736));
#104573=CARTESIAN_POINT('Ctrl Pts',(-18.5230658965378,21.3175812657428,
-14.2998364357305));
#104574=CARTESIAN_POINT('Ctrl Pts',(-18.7299334077737,21.3361152662931,
-14.2877568201063));
#104575=CARTESIAN_POINT('Ctrl Pts',(-18.9161494182181,21.3282999399898,
-14.2778298586475));
#104576=CARTESIAN_POINT('Ctrl Pts',(-19.2067678941241,21.2774353700723,
-14.2617461892765));
#104577=CARTESIAN_POINT('Ctrl Pts',(-19.3129236077801,21.2502414434953,
-14.255713645448));
#104578=CARTESIAN_POINT('Ctrl Pts',(-19.4276535289006,21.2111682311234,
-14.2485600409417));
#104579=CARTESIAN_POINT('Ctrl Pts',(-19.4387884746274,21.2072718659285,
-14.2478588884412));
#104580=CARTESIAN_POINT('Ctrl Pts',(-19.4545987856627,21.2015907228319,
-14.2468527465442));
#104581=CARTESIAN_POINT('Ctrl Pts',(-19.4593015164607,21.1998820339005,
-14.2465521309908));
#104582=CARTESIAN_POINT('Ctrl Pts',(-19.4674056668768,21.1969049086939,
-14.246031694697));
#104583=CARTESIAN_POINT('Ctrl Pts',(-19.4708099975528,21.195644352508,-14.2458123430376));
#104584=CARTESIAN_POINT('Ctrl Pts',(-19.4774125708833,21.1931802205314,
-14.2453854722866));
#104585=CARTESIAN_POINT('Ctrl Pts',(-19.4806111475846,21.1919776553842,
-14.245178019509));
#104586=CARTESIAN_POINT('Ctrl Pts',(-19.489250696036,21.1887055578311,-14.2446159245346));
#104587=CARTESIAN_POINT('Ctrl Pts',(-19.4946860188193,21.1866213367628,
-14.2442604157527));
#104588=CARTESIAN_POINT('Ctrl Pts',(-19.514929398964,21.1787629163425,-14.2429295063666));
#104589=CARTESIAN_POINT('Ctrl Pts',(-19.529680450471,21.1728445930577,-14.2419459861255));
#104590=CARTESIAN_POINT('Ctrl Pts',(-19.6585595515571,21.1194439722711,
-14.2332409824132));
#104591=CARTESIAN_POINT('Ctrl Pts',(-19.7683817729444,21.0622205094752,
-14.2250614637882));
#104592=CARTESIAN_POINT('Ctrl Pts',(-20.0134987630084,20.9058493352509,
-14.2058482408526));
#104593=CARTESIAN_POINT('Ctrl Pts',(-20.1433070245278,20.799554649955,-14.1949304646484));
#104594=CARTESIAN_POINT('Ctrl Pts',(-20.2740376622133,20.6637306971835,
-14.1833518380511));
#104595=CARTESIAN_POINT('Ctrl Pts',(-20.2885731834927,20.6481655258684,
-14.1820539067332));
#104596=CARTESIAN_POINT('Ctrl Pts',(-20.3089101436537,20.6257183189353,
-14.1802221201685));
#104597=CARTESIAN_POINT('Ctrl Pts',(-20.3149060239489,20.6190149252966,
-14.1796800407352));
#104598=CARTESIAN_POINT('Ctrl Pts',(-20.3251769992412,20.6073836548643,
-14.1787478709533));
#104599=CARTESIAN_POINT('Ctrl Pts',(-20.3294723330081,20.6024738914441,
-14.1783569353496));
#104600=CARTESIAN_POINT('Ctrl Pts',(-20.3376537895791,20.593034421189,-14.1776101519217));
#104601=CARTESIAN_POINT('Ctrl Pts',(-20.3415435794725,20.5885079888707,
-14.177254153898));
#104602=CARTESIAN_POINT('Ctrl Pts',(-20.3516099194524,20.5766933820188,
-14.1763303528689));
#104603=CARTESIAN_POINT('Ctrl Pts',(-20.3577564141384,20.569379688192,-14.1757637884633));
#104604=CARTESIAN_POINT('Ctrl Pts',(-20.3785534567884,20.5442904860486,
-14.1738379611169));
#104605=CARTESIAN_POINT('Ctrl Pts',(-20.3929636275252,20.5263171998545,
-14.172488428772));
#104606=CARTESIAN_POINT('Ctrl Pts',(-20.5142339457141,20.3698968294222,
-14.1609878779454));
#104607=CARTESIAN_POINT('Ctrl Pts',(-20.6038503965437,20.2189389781553,
-14.1515818203584));
#104608=CARTESIAN_POINT('Ctrl Pts',(-20.7088877048325,19.9785607387108,
-14.1373097913567));
#104609=CARTESIAN_POINT('Ctrl Pts',(-20.7388927332316,19.8963711717698,
-14.1325253074778));
#104610=CARTESIAN_POINT('Ctrl Pts',(-20.774507313731,19.7762056476618,-14.1253702987708));
#104611=CARTESIAN_POINT('Ctrl Pts',(-20.7843050112086,19.7395607630782,
-14.1231673499135));
#104612=CARTESIAN_POINT('Ctrl Pts',(-20.7948724782272,19.6953047074352,
-14.1204602440323));
#104613=CARTESIAN_POINT('Ctrl Pts',(-20.7965927840851,19.6879249671223,
-14.1200072897686));
#104614=CARTESIAN_POINT('Ctrl Pts',(-20.7992012898457,19.676456909532,-14.1193007881222));
#104615=CARTESIAN_POINT('Ctrl Pts',(-20.8001170725569,19.6723748411057,
-14.1190487952217));
#104616=CARTESIAN_POINT('Ctrl Pts',(-20.8017905255752,19.6648105795938,
-14.1185808466496));
#104617=CARTESIAN_POINT('Ctrl Pts',(-20.8025515054841,19.6613291778122,
-14.1183650833212));
#104618=CARTESIAN_POINT('Ctrl Pts',(-20.8042489796066,19.6534683252953,
-14.1178770167999));
#104619=CARTESIAN_POINT('Ctrl Pts',(-20.8051803639459,19.6490878400551,
-14.1176044271311));
#104620=CARTESIAN_POINT('Ctrl Pts',(-20.8078797709372,19.6361909583271,
-14.1168001423127));
#104621=CARTESIAN_POINT('Ctrl Pts',(-20.8096091896308,19.6276667029089,
-14.1162663232883));
#104622=CARTESIAN_POINT('Ctrl Pts',(-20.8214936993915,19.5671776614161,
-14.1124637251107));
#104623=CARTESIAN_POINT('Ctrl Pts',(-20.8297477800314,19.5148629594319,
-14.1090993050803));
#104624=CARTESIAN_POINT('Ctrl Pts',(-20.8378088383535,19.4474349197908,
-14.1047116242331));
#104625=CARTESIAN_POINT('Ctrl Pts',(-20.8394281081353,19.4325526253307,
-14.103739991965));
#104626=CARTESIAN_POINT('Ctrl Pts',(-20.8475637100768,19.3496083921713,
-14.0983109135824));
#104627=CARTESIAN_POINT('Ctrl Pts',(-20.8509374101805,19.2812805401817,
-14.0937882933207));
#104628=CARTESIAN_POINT('Ctrl Pts',(-20.8511442879771,19.0521414075599,
-14.0786473323232));
#104629=CARTESIAN_POINT('Ctrl Pts',(-20.8329752264163,18.8918491684336,
-14.068149332205));
#104630=CARTESIAN_POINT('Ctrl Pts',(-20.7914795967818,18.711968850762,-14.0567778297863));
#104631=CARTESIAN_POINT('Ctrl Pts',(-20.7857446857667,18.688890628449,-14.0553255502215));
#104632=CARTESIAN_POINT('Ctrl Pts',(-20.7771304028878,18.6565626300262,
-14.0532998512992));
#104633=CARTESIAN_POINT('Ctrl Pts',(-20.7745746989702,18.6472291749167,
-14.0527160284796));
#104634=CARTESIAN_POINT('Ctrl Pts',(-20.7703333352122,18.6321464466819,
-14.0517741466886));
#104635=CARTESIAN_POINT('Ctrl Pts',(-20.7686871311575,18.6263863089748,
-14.0514148108242));
#104636=CARTESIAN_POINT('Ctrl Pts',(-20.7652024820197,18.6143863980278,
-14.0506669636328));
#104637=CARTESIAN_POINT('Ctrl Pts',(-20.7633596813769,18.608147946773,-14.050278598788));
#104638=CARTESIAN_POINT('Ctrl Pts',(-20.758930467693,18.593404154119,-14.0493616993591));
#104639=CARTESIAN_POINT('Ctrl Pts',(-20.7563191638836,18.5849063720951,
-14.0488339846072));
#104640=CARTESIAN_POINT('Ctrl Pts',(-20.7474528177427,18.5566875481663,
-14.0470839024837));
#104641=CARTESIAN_POINT('Ctrl Pts',(-20.740962098308,18.5370413850976,-14.0458692713577));
#104642=CARTESIAN_POINT('Ctrl Pts',(-20.7304048691224,18.5065926607223,
-14.0439913314941));
#104643=CARTESIAN_POINT('Ctrl Pts',(-20.7265368450947,18.4957245523086,
-14.0433219475054));
#104644=CARTESIAN_POINT('Ctrl Pts',(-20.7225806179957,18.4848897289449,
-14.042655348398));
#104645=CARTESIAN_POINT('Origin',(-18.734,19.211,0.));
#104646=CARTESIAN_POINT('',(-20.7225806137986,18.4848897174502,-13.2445592988469));
#104647=CARTESIAN_POINT('',(-20.722580578415,18.4848896205462,-13.4647888589437));
#104648=CARTESIAN_POINT('',(-20.7225806137986,18.4848897174502,0.));
#104649=CARTESIAN_POINT('',(-20.8509991049198,19.2090532671894,-13.5109437209775));
#104650=CARTESIAN_POINT('Ctrl Pts',(-20.722580578415,18.4848896205462,-13.4647888589437));
#104651=CARTESIAN_POINT('Ctrl Pts',(-20.7382333493556,18.5277574780669,
-13.4673502679699));
#104652=CARTESIAN_POINT('Ctrl Pts',(-20.7525027540004,18.5711391169453,
-13.469956309288));
#104653=CARTESIAN_POINT('Ctrl Pts',(-20.7697993266343,18.630088286143,-13.4735579249014));
#104654=CARTESIAN_POINT('Ctrl Pts',(-20.7740668388379,18.6452574987151,
-13.4744900199622));
#104655=CARTESIAN_POINT('Ctrl Pts',(-20.7796729209201,18.6660734476574,
-13.4757780950466));
#104656=CARTESIAN_POINT('Ctrl Pts',(-20.7811583220313,18.6716805681512,
-13.4761259490076));
#104657=CARTESIAN_POINT('Ctrl Pts',(-20.7834811070311,18.6805965296512,
-13.476680591069));
#104658=CARTESIAN_POINT('Ctrl Pts',(-20.7843335776018,18.6839014611929,
-13.4768865132768));
#104659=CARTESIAN_POINT('Ctrl Pts',(-20.7860768721339,18.6907282364931,
-13.4773125806241));
#104660=CARTESIAN_POINT('Ctrl Pts',(-20.786966621664,18.6942503056574,-13.4775327886363));
#104661=CARTESIAN_POINT('Ctrl Pts',(-20.7890638353797,18.7026430250298,
-13.4780584284453));
#104662=CARTESIAN_POINT('Ctrl Pts',(-20.7902630515217,18.7075156971233,
-13.4783643314232));
#104663=CARTESIAN_POINT('Ctrl Pts',(-20.7927674039711,18.7178496121134,
-13.4790145549943));
#104664=CARTESIAN_POINT('Ctrl Pts',(-20.7940681569147,18.7233118660594,
-13.4793591136575));
#104665=CARTESIAN_POINT('Ctrl Pts',(-20.7975804759611,18.7383259597019,
-13.4803084562977));
#104666=CARTESIAN_POINT('Ctrl Pts',(-20.7997474095153,18.7478879604707,
-13.4809155631972));
#104667=CARTESIAN_POINT('Ctrl Pts',(-20.8343835380824,18.9058077632302,
-13.4909794453464));
#104668=CARTESIAN_POINT('Ctrl Pts',(-20.8508585305076,19.0572035887683,
-13.5011356069027));
#104669=CARTESIAN_POINT('Ctrl Pts',(-20.8509990928573,19.2090401934883,
-13.5111420888258));
#104670=CARTESIAN_POINT('Ctrl Pts',(-20.8509991049198,19.2090532671894,
-13.5109437209775));
#104671=CARTESIAN_POINT('Ctrl Pts',(-20.8510652701871,19.2810055201563,
-13.5152699622426));
#104672=CARTESIAN_POINT('Ctrl Pts',(-20.84745892973,19.3530526998716,-13.5195962035077));
#104673=CARTESIAN_POINT('Ctrl Pts',(-20.8401777557621,19.424785549402,-13.5239224447729));
#104674=CARTESIAN_POINT('Ctrl Pts',(-20.8329012160598,19.4964727429599,
-13.5282459325052));
#104675=CARTESIAN_POINT('Ctrl Pts',(-20.8219545300652,19.5678455121802,
-13.5325694202376));
#104676=CARTESIAN_POINT('Ctrl Pts',(-20.8073873938026,19.6384970353352,
-13.5368929079699));
#104677=CARTESIAN_POINT('Ctrl Pts',(-20.7928244565269,19.7091281931407,
-13.541215149454));
#104678=CARTESIAN_POINT('Ctrl Pts',(-20.7746432396996,19.7790380332555,
-13.5455373909381));
#104679=CARTESIAN_POINT('Ctrl Pts',(-20.7529446959791,19.8478291093989,
-13.5498596324221));
#104680=CARTESIAN_POINT('Ctrl Pts',(-20.7312448511872,19.91662431034,-13.5541821330731));
#104681=CARTESIAN_POINT('Ctrl Pts',(-20.7060274126677,19.9843001434093,
-13.5585046337241));
#104682=CARTESIAN_POINT('Ctrl Pts',(-20.6774428750096,20.0504753073047,
-13.5628271343751));
#104683=CARTESIAN_POINT('Ctrl Pts',(-20.6488284904874,20.1167195687362,
-13.5671541484135));
#104684=CARTESIAN_POINT('Ctrl Pts',(-20.6168401898343,20.1814595804048,
-13.5714811624518));
#104685=CARTESIAN_POINT('Ctrl Pts',(-20.5816757716208,20.2443359777756,
-13.5758081764901));
#104686=CARTESIAN_POINT('Ctrl Pts',(-20.5464899011033,20.3072507333408,
-13.5801378302542));
#104687=CARTESIAN_POINT('Ctrl Pts',(-20.5081243239342,20.3682991960122,
-13.5844674840182));
#104688=CARTESIAN_POINT('Ctrl Pts',(-20.4668202589893,20.4271508747011,
-13.5887971377823));
#104689=CARTESIAN_POINT('Ctrl Pts',(-20.4254474059594,20.4861005653963,
-13.5931340021827));
#104690=CARTESIAN_POINT('Ctrl Pts',(-20.3811266092583,20.5428457872319,
-13.5974708665831));
#104691=CARTESIAN_POINT('Ctrl Pts',(-20.334138776401,20.5970897865066,-13.6018077309835));
#104692=CARTESIAN_POINT('Ctrl Pts',(-20.317565474994,20.6162224447893,-13.6033374069975));
#104693=CARTESIAN_POINT('Ctrl Pts',(-20.3006606978845,20.6350442778647,
-13.6048670830114));
#104694=CARTESIAN_POINT('Ctrl Pts',(-20.2834377820479,20.6535434342032,
-13.6063967590254));
#104695=CARTESIAN_POINT('Ctrl Pts',(-20.2340300954521,20.7066122947448,
-13.6107849679563));
#104696=CARTESIAN_POINT('Ctrl Pts',(-20.1817963672775,20.757243459066,-13.6151731768872));
#104697=CARTESIAN_POINT('Ctrl Pts',(-20.1270066890246,20.8051208750696,
-13.6195613858181));
#104698=CARTESIAN_POINT('Ctrl Pts',(-20.0722983277385,20.8529272330497,
-13.6239430819193));
#104699=CARTESIAN_POINT('Ctrl Pts',(-20.0150419071299,20.8979876412174,
-13.6283247780206));
#104700=CARTESIAN_POINT('Ctrl Pts',(-19.9555455237305,20.9400215537853,
-13.6327064741219));
#104701=CARTESIAN_POINT('Ctrl Pts',(-19.8961190533166,20.9820060731606,
-13.6370830213815));
#104702=CARTESIAN_POINT('Ctrl Pts',(-19.834458240882,21.0209708847355,-13.6414595686412));
#104703=CARTESIAN_POINT('Ctrl Pts',(-19.7709042257781,21.0566756558408,
-13.6458361159008));
#104704=CARTESIAN_POINT('Ctrl Pts',(-19.7073905157069,21.0923577834992,
-13.6502098876178));
#104705=CARTESIAN_POINT('Ctrl Pts',(-19.6419864047143,21.1247837371303,
-13.6545836593348));
#104706=CARTESIAN_POINT('Ctrl Pts',(-19.5750607832518,21.1537572568069,
-13.6589574310518));
#104707=CARTESIAN_POINT('Ctrl Pts',(-19.5081555274806,21.1827219597441,
-13.6633298718153));
#104708=CARTESIAN_POINT('Ctrl Pts',(-19.4397301228475,21.2082361229382,
-13.6677023125789));
#104709=CARTESIAN_POINT('Ctrl Pts',(-19.3701752330585,21.2301508296417,
-13.6720747533424));
#104710=CARTESIAN_POINT('Ctrl Pts',(-19.3006185647433,21.2520660967068,
-13.6764473059098));
#104711=CARTESIAN_POINT('Ctrl Pts',(-19.2299328146144,21.2703815814965,
-13.6808198584771));
#104712=CARTESIAN_POINT('Ctrl Pts',(-19.1585240564091,21.2849981498376,
-13.6851924110445));
#104713=CARTESIAN_POINT('Ctrl Pts',(-19.0870411875011,21.2996298878047,
-13.6895695016118));
#104714=CARTESIAN_POINT('Ctrl Pts',(-19.0148342859528,21.3105549478118,
-13.6939465921791));
#104715=CARTESIAN_POINT('Ctrl Pts',(-18.94231905461,21.3177254618213,-13.6983236827465));
#104716=CARTESIAN_POINT('Ctrl Pts',(-18.869764220008,21.3248998919147,-13.7027031638054));
#104717=CARTESIAN_POINT('Ctrl Pts',(-18.7969012025304,21.3283156708867,
-13.7070826448644));
#104718=CARTESIAN_POINT('Ctrl Pts',(-18.7241475303624,21.3279770732915,
-13.7114621259233));
#104719=CARTESIAN_POINT('Ctrl Pts',(-18.6512649027988,21.3276378755344,
-13.715849369583));
#104720=CARTESIAN_POINT('Ctrl Pts',(-18.5784924896188,21.3235310394329,
-13.7202366132427));
#104721=CARTESIAN_POINT('Ctrl Pts',(-18.5062439309,21.3157128481073,-13.7246238569025));
#104722=CARTESIAN_POINT('Ctrl Pts',(-18.4571218728267,21.3103972313652,
-13.7276067598372));
#104723=CARTESIAN_POINT('Ctrl Pts',(-18.408241843935,21.3033670563133,-13.730589662772));
#104724=CARTESIAN_POINT('Ctrl Pts',(-18.3597305432933,21.2946533717911,
-13.7335725657068));
#104725=CARTESIAN_POINT('Ctrl Pts',(-18.2883645862437,21.2818344939807,
-13.7379607746377));
#104726=CARTESIAN_POINT('Ctrl Pts',(-18.2175186632351,21.2653198837036,
-13.7423489835686));
#104727=CARTESIAN_POINT('Ctrl Pts',(-18.1476047194716,21.2451655721632,
-13.7467371924995));
#104728=CARTESIAN_POINT('Ctrl Pts',(-18.0777945395925,21.2250411729628,
-13.7511188886007));
#104729=CARTESIAN_POINT('Ctrl Pts',(-18.0089140527663,21.201287928559,-13.755500584702));
#104730=CARTESIAN_POINT('Ctrl Pts',(-17.9413659204117,21.1740130452636,
-13.7598822808033));
#104731=CARTESIAN_POINT('Ctrl Pts',(-17.8738971624885,21.1467702121269,
-13.7642588280629));
#104732=CARTESIAN_POINT('Ctrl Pts',(-17.8077580939881,21.116014140384,-13.7686353753226));
#104733=CARTESIAN_POINT('Ctrl Pts',(-17.7433354489126,21.0819015867273,
-13.7730119225822));
#104734=CARTESIAN_POINT('Ctrl Pts',(-17.6789536597423,21.0478106667564,
-13.7773856942992));
#104735=CARTESIAN_POINT('Ctrl Pts',(-17.6162865594638,21.0103677135303,
-13.7817594660161));
#104736=CARTESIAN_POINT('Ctrl Pts',(-17.5556988450219,20.9697766737642,
-13.7861332377331));
#104737=CARTESIAN_POINT('Ctrl Pts',(-17.4951295676249,20.9291979859878,
-13.7905056784967));
#104738=CARTESIAN_POINT('Ctrl Pts',(-17.4366388203451,20.885473381869,-13.7948781192602));
#104739=CARTESIAN_POINT('Ctrl Pts',(-17.380563277455,20.8388507419498,-13.7992505600238));
#104740=CARTESIAN_POINT('Ctrl Pts',(-17.3244863007071,20.7922269098846,
-13.8036231125911));
#104741=CARTESIAN_POINT('Ctrl Pts',(-17.2708250206039,20.7427052048249,
-13.8079956651585));
#104742=CARTESIAN_POINT('Ctrl Pts',(-17.2198825933089,20.6905734110732,
-13.8123682177258));
#104743=CARTESIAN_POINT('Ctrl Pts',(-17.1688872960413,20.6383875129797,
-13.8167453082932));
#104744=CARTESIAN_POINT('Ctrl Pts',(-17.1206168232076,20.5835864635392,
-13.8211223988605));
#104745=CARTESIAN_POINT('Ctrl Pts',(-17.0753364363183,20.5264938929979,
-13.8254994894278));
#104746=CARTESIAN_POINT('Ctrl Pts',(-17.0300313201292,20.4693701420848,
-13.8298789704868));
#104747=CARTESIAN_POINT('Ctrl Pts',(-16.9877198211683,20.409952771581,-13.8342584515457));
#104748=CARTESIAN_POINT('Ctrl Pts',(-16.9486243452996,20.3485951703497,
-13.8386379326047));
#104749=CARTESIAN_POINT('Ctrl Pts',(-16.9094595729623,20.2871288131822,
-13.8430251762644));
#104750=CARTESIAN_POINT('Ctrl Pts',(-16.8735224451864,20.2237157776925,
-13.8474124199241));
#104751=CARTESIAN_POINT('Ctrl Pts',(-16.8409895323034,20.1587343347116,
-13.8517996635838));
#104752=CARTESIAN_POINT('Ctrl Pts',(-16.8188702864072,20.1145532150819,
-13.8547825665186));
#104753=CARTESIAN_POINT('Ctrl Pts',(-16.7983237185204,20.0696475457982,
-13.8577654694534));
#104754=CARTESIAN_POINT('Ctrl Pts',(-16.7793923012851,20.0241406668741,
-13.8607483723882));
#104755=CARTESIAN_POINT('Ctrl Pts',(-16.7515419099038,19.9571945754736,
-13.8651365813191));
#104756=CARTESIAN_POINT('Ctrl Pts',(-16.7270805292279,19.8886853205153,
-13.86952479025));
#104757=CARTESIAN_POINT('Ctrl Pts',(-16.706184024008,19.8189896113517,-13.8739129991809));
#104758=CARTESIAN_POINT('Ctrl Pts',(-16.6853185326666,19.7493973421762,
-13.8782946952822));
#104759=CARTESIAN_POINT('Ctrl Pts',(-16.6680075510805,19.6786225726489,
-13.8826763913834));
#104760=CARTESIAN_POINT('Ctrl Pts',(-16.6543788886961,19.6070619060438,
-13.8870580874847));
#104761=CARTESIAN_POINT('Ctrl Pts',(-16.6407662410746,19.5355853289171,
-13.8914346347443));
#104762=CARTESIAN_POINT('Ctrl Pts',(-16.6308274068039,19.4633251607434,
-13.895811182004));
#104763=CARTESIAN_POINT('Ctrl Pts',(-16.6246399100932,19.390691433041,-13.9001877292636));
#104764=CARTESIAN_POINT('Ctrl Pts',(-16.618456337403,19.318103768593,-13.9045615009806));
#104765=CARTESIAN_POINT('Ctrl Pts',(-16.6160194227851,19.2451434941229,
-13.9089352726976));
#104766=CARTESIAN_POINT('Ctrl Pts',(-16.6173550828665,19.1722276545356,
-13.9133090444145));
#104767=CARTESIAN_POINT('Ctrl Pts',(-16.618690336502,19.099334003483,-13.9176814851781));
#104768=CARTESIAN_POINT('Ctrl Pts',(-16.6237958768595,19.0264852424754,
-13.9220539259417));
#104769=CARTESIAN_POINT('Ctrl Pts',(-16.6326455110292,18.9540986343319,
-13.9264263667052));
#104770=CARTESIAN_POINT('Ctrl Pts',(-16.6414953714849,18.8817101752551,
-13.9307989192725));
#104771=CARTESIAN_POINT('Ctrl Pts',(-16.6540894553072,18.8097843710746,
-13.9351714718399));
#104772=CARTESIAN_POINT('Ctrl Pts',(-16.6703498741218,18.7387319003334,
-13.9395440244072));
#104773=CARTESIAN_POINT('Ctrl Pts',(-16.6866271686123,18.6676056886579,
-13.9439211149745));
#104774=CARTESIAN_POINT('Ctrl Pts',(-16.7065782873147,18.5973550912947,
-13.9482982055419));
#104775=CARTESIAN_POINT('Ctrl Pts',(-16.7300746894319,18.5283783261097,
-13.9526752961092));
#104776=CARTESIAN_POINT('Ctrl Pts',(-16.7535839238065,18.4593638901532,
-13.9570547771681));
#104777=CARTESIAN_POINT('Ctrl Pts',(-16.7806421175109,18.3916251197528,
-13.9614342582271));
#104778=CARTESIAN_POINT('Ctrl Pts',(-16.811072510512,18.325540305733,-13.965813739286));
#104779=CARTESIAN_POINT('Ctrl Pts',(-16.8415568411804,18.2593383568239,
-13.9702009829457));
#104780=CARTESIAN_POINT('Ctrl Pts',(-16.8754250830332,18.1947966461509,
-13.9745882266055));
#104781=CARTESIAN_POINT('Ctrl Pts',(-16.9124547443357,18.1322683922463,
-13.9789754702652));
#104782=CARTESIAN_POINT('Ctrl Pts',(-16.9376313458519,18.0897552047992,
-13.9819583732));
#104783=CARTESIAN_POINT('Ctrl Pts',(-16.9642684397429,18.0481722056908,
-13.9849412761348));
#104784=CARTESIAN_POINT('Ctrl Pts',(-16.992285306212,18.0076218693017,-13.9879241790697));
#104785=CARTESIAN_POINT('Ctrl Pts',(-17.033501486001,17.9479674480279,-13.9923123880006));
#104786=CARTESIAN_POINT('Ctrl Pts',(-17.0778664461833,17.8903165376486,
-13.9967005969315));
#104787=CARTESIAN_POINT('Ctrl Pts',(-17.1251586260628,17.8350209182157,
-14.0010888058624));
#104788=CARTESIAN_POINT('Ctrl Pts',(-17.1723806165062,17.7798073666503,
-14.0054705019636));
#104789=CARTESIAN_POINT('Ctrl Pts',(-17.2225208913247,17.7269425302633,
-14.0098521980649));
#104790=CARTESIAN_POINT('Ctrl Pts',(-17.2753151507578,17.6767485504028,
-14.0142338941661));
#104791=CARTESIAN_POINT('Ctrl Pts',(-17.3280473727346,17.6266135524631,
-14.0186104414258));
#104792=CARTESIAN_POINT('Ctrl Pts',(-17.3834270362633,17.5791435071861,
-14.0229869886854));
#104793=CARTESIAN_POINT('Ctrl Pts',(-17.4411513321101,17.5346255424472,
-14.0273635359451));
#104794=CARTESIAN_POINT('Ctrl Pts',(-17.4988390200475,17.4901358103546,
-14.031737307662));
#104795=CARTESIAN_POINT('Ctrl Pts',(-17.5588680090001,17.4485947380414,
-14.036111079379));
#104796=CARTESIAN_POINT('Ctrl Pts',(-17.6209016583806,17.4102498557867,
-14.040484851096));
#104797=CARTESIAN_POINT('Ctrl Pts',(-17.6829164307132,17.3719166420085,
-14.0448572918595));
#104798=CARTESIAN_POINT('Ctrl Pts',(-17.7469342423155,17.3367779408325,
-14.0492297326231));
#104799=CARTESIAN_POINT('Ctrl Pts',(-17.8125900634645,17.3050375846167,
-14.0536021733866));
#104800=CARTESIAN_POINT('Ctrl Pts',(-17.87824756344,17.2732964167966,-14.057974725954));
#104801=CARTESIAN_POINT('Ctrl Pts',(-17.9455427209579,17.244953974612,-14.0623472785213));
#104802=CARTESIAN_POINT('Ctrl Pts',(-18.0140880608552,17.2201670587724,
-14.0667198310887));
#104803=CARTESIAN_POINT('Ctrl Pts',(-18.0827045396917,17.1953544181367,
-14.071096921656));
#104804=CARTESIAN_POINT('Ctrl Pts',(-18.1525733368268,17.1741048356876,
-14.0754740122233));
#104805=CARTESIAN_POINT('Ctrl Pts',(-18.2232900373592,17.1565257767352,
-14.0798511027906));
#104806=CARTESIAN_POINT('Ctrl Pts',(-18.2940453589065,17.1389371172062,
-14.0842305838496));
#104807=CARTESIAN_POINT('Ctrl Pts',(-18.3656490319735,17.1250230644093,
-14.0886100649085));
#104808=CARTESIAN_POINT('Ctrl Pts',(-18.4376872969892,17.1148397527779,
-14.0929895459675));
#104809=CARTESIAN_POINT('Ctrl Pts',(-18.5098532493459,17.1046383912949,
-14.0973767896272));
#104810=CARTESIAN_POINT('Ctrl Pts',(-18.5824548510276,17.0981810190706,
-14.1017640332869));
#104811=CARTESIAN_POINT('Ctrl Pts',(-18.6550746705905,17.0954717462587,
-14.1061512769466));
#104812=CARTESIAN_POINT('Ctrl Pts',(-18.7044491502642,17.0936297018115,
-14.1091341798814));
#104813=CARTESIAN_POINT('Ctrl Pts',(-18.7538320255728,17.093519193629,-14.1121170828162));
#104814=CARTESIAN_POINT('Ctrl Pts',(-18.8030934396837,17.0951278165748,
-14.1150999857511));
#104815=CARTESIAN_POINT('Ctrl Pts',(-18.8755629038515,17.0974942943756,
-14.119488194682));
#104816=CARTESIAN_POINT('Ctrl Pts',(-18.9480521075248,17.1035928606293,
-14.1238764036129));
#104817=CARTESIAN_POINT('Ctrl Pts',(-19.0201453327482,17.1134276297237,
-14.1282646125438));
#104818=CARTESIAN_POINT('Ctrl Pts',(-19.0921315596719,17.1232478023901,
-14.132646308645));
#104819=CARTESIAN_POINT('Ctrl Pts',(-19.1637225008055,17.1367931053666,
-14.1370280047463));
#104820=CARTESIAN_POINT('Ctrl Pts',(-19.2345042258075,17.1540156733828,
-14.1414097008476));
#104821=CARTESIAN_POINT('Ctrl Pts',(-19.3052027766498,17.171218003511,-14.1457862481072));
#104822=CARTESIAN_POINT('Ctrl Pts',(-19.37509353394,17.1920889013491,-14.1501627953669));
#104823=CARTESIAN_POINT('Ctrl Pts',(-19.4437711636788,17.2165291691253,
-14.1545393426265));
#104824=CARTESIAN_POINT('Ctrl Pts',(-19.512405239063,17.2409539372389,-14.1589131143435));
#104825=CARTESIAN_POINT('Ctrl Pts',(-19.5798272600414,17.2689434226003,
-14.1632868860605));
#104826=CARTESIAN_POINT('Ctrl Pts',(-19.6456468756569,17.3003485471952,
-14.1676606577774));
#104827=CARTESIAN_POINT('Ctrl Pts',(-19.7114464621424,17.3317441151053,
-14.172033098541));
#104828=CARTESIAN_POINT('Ctrl Pts',(-19.775644176238,17.3665530511362,-14.1764055393046));
#104829=CARTESIAN_POINT('Ctrl Pts',(-19.837871043522,17.4045787536475,-14.1807779800681));
#104830=CARTESIAN_POINT('Ctrl Pts',(-19.9000995019538,17.4426054284802,
-14.1851505326355));
#104831=CARTESIAN_POINT('Ctrl Pts',(-19.9603566029532,17.4838487798657,
-14.1895230852028));
#104832=CARTESIAN_POINT('Ctrl Pts',(-20.018300768981,17.5280678757612,-14.1938956377702));
#104833=CARTESIAN_POINT('Ctrl Pts',(-20.0763050716499,17.5723328639025,
-14.1982727283375));
#104834=CARTESIAN_POINT('Ctrl Pts',(-20.131991262393,17.6195794693668,-14.2026498189048));
#104835=CARTESIAN_POINT('Ctrl Pts',(-20.1850500777755,17.6695258121565,
-14.2070269094722));
#104836=CARTESIAN_POINT('Ctrl Pts',(-20.2381378705463,17.7194994324977,
-14.2114063905311));
#104837=CARTESIAN_POINT('Ctrl Pts',(-20.2885950971619,17.772175377142,-14.21578587159));
#104838=CARTESIAN_POINT('Ctrl Pts',(-20.3361505972391,17.8272361242732,
-14.220165352649));
#104839=CARTESIAN_POINT('Ctrl Pts',(-20.383790389121,17.8823944662092,-14.2245525963087));
#104840=CARTESIAN_POINT('Ctrl Pts',(-20.4285178872523,17.9399456706598,
-14.2289398399684));
#104841=CARTESIAN_POINT('Ctrl Pts',(-20.470103687921,17.9995409685891,-14.2333270836282));
#104842=CARTESIAN_POINT('Ctrl Pts',(-20.4983780251772,18.0400600285913,
-14.2363099865629));
#104843=CARTESIAN_POINT('Ctrl Pts',(-20.5252009588543,18.0815233957326,
-14.2392928894977));
#104844=CARTESIAN_POINT('Ctrl Pts',(-20.5505126306683,18.1238151663023,
-14.2422757924325));
#104845=CARTESIAN_POINT('Ctrl Pts',(-20.5890177730692,18.1881511240427,
-14.2468135054337));
#104846=CARTESIAN_POINT('Ctrl Pts',(-20.6241652163586,18.2546416816847,
-14.2513512184349));
#104847=CARTESIAN_POINT('Ctrl Pts',(-20.6557165770165,18.3229153206929,
-14.255888931436));
#104848=CARTESIAN_POINT('Ctrl Pts',(-20.680200416808,18.37589562977,-14.2594101944124));
#104849=CARTESIAN_POINT('Ctrl Pts',(-20.7025195409889,18.4299489440717,
-14.2629314573889));
#104850=CARTESIAN_POINT('Ctrl Pts',(-20.7225806137986,18.4848897174502,
-14.2664527203653));
#104851=CARTESIAN_POINT('',(-20.8509999987372,19.2109341274623,-13.2889033777666));
#104852=CARTESIAN_POINT('Ctrl Pts',(-20.7225806179957,18.4848897289449,
-14.042655348398));
#104853=CARTESIAN_POINT('Ctrl Pts',(-20.6958130730314,18.411582101675,-14.0381451872939));
#104854=CARTESIAN_POINT('Ctrl Pts',(-20.6650078049974,18.3397979900317,
-14.0337656578687));
#104855=CARTESIAN_POINT('Ctrl Pts',(-20.5703572068461,18.1490855410707,
-14.0220205677548));
#104856=CARTESIAN_POINT('Ctrl Pts',(-20.4990149242829,18.0343138383552,
-14.0148421229976));
#104857=CARTESIAN_POINT('Ctrl Pts',(-20.3708541763278,17.8662886020928,
-14.0031498605669));
#104858=CARTESIAN_POINT('Ctrl Pts',(-20.3212057311274,17.808033269361,-13.9988302806948));
#104859=CARTESIAN_POINT('Ctrl Pts',(-20.2619779462149,17.7457141564181,
-13.9937349088717));
#104860=CARTESIAN_POINT('Ctrl Pts',(-20.2553888180463,17.7388738966237,
-13.9931687790576));
#104861=CARTESIAN_POINT('Ctrl Pts',(-20.2455537543989,17.7288005419894,
-13.9923244195925));
#104862=CARTESIAN_POINT('Ctrl Pts',(-20.2423428873456,17.7255331646068,
-13.9920488627986));
#104863=CARTESIAN_POINT('Ctrl Pts',(-20.2366096472776,17.7197367750051,
-13.9915569605736));
#104864=CARTESIAN_POINT('Ctrl Pts',(-20.2340914540627,17.7172036994518,
-13.991340944181));
#104865=CARTESIAN_POINT('Ctrl Pts',(-20.228661806659,17.7117695387174,-13.9908752471347));
#104866=CARTESIAN_POINT('Ctrl Pts',(-20.2257483539505,17.7088705980691,
-13.9906254109197));
#104867=CARTESIAN_POINT('Ctrl Pts',(-20.2176786501626,17.7008877204961,
-13.9899335952082));
#104868=CARTESIAN_POINT('Ctrl Pts',(-20.2125047848917,17.6958217823571,
-13.9894902443921));
#104869=CARTESIAN_POINT('Ctrl Pts',(-20.1839451579348,17.6681434754153,
-13.9870446022492));
#104870=CARTESIAN_POINT('Ctrl Pts',(-20.1600679286851,17.6460472178848,
-13.9850059843469));
#104871=CARTESIAN_POINT('Ctrl Pts',(-20.0137580372223,17.5167796681214,
-13.9726001129272));
#104872=CARTESIAN_POINT('Ctrl Pts',(-19.8798138254873,17.4234671266425,
-13.9616428496239));
#104873=CARTESIAN_POINT('Ctrl Pts',(-19.633621638164,17.2911002983456,-13.9433847645602));
#104874=CARTESIAN_POINT('Ctrl Pts',(-19.5263234271556,17.2443873413246,
-13.935943923391));
#104875=CARTESIAN_POINT('Ctrl Pts',(-19.4021738970265,17.2021603277574,
-13.9279368651318));
#104876=CARTESIAN_POINT('Ctrl Pts',(-19.3885991772499,17.1976959697293,
-13.9270688889833));
#104877=CARTESIAN_POINT('Ctrl Pts',(-19.3669223603483,17.1908094731998,
-13.9256945802473));
#104878=CARTESIAN_POINT('Ctrl Pts',(-19.3588493390738,17.1882978999614,
-13.9251853195911));
#104879=CARTESIAN_POINT('Ctrl Pts',(-19.3445847673627,17.1839536435782,
-13.9242899413779));
#104880=CARTESIAN_POINT('Ctrl Pts',(-19.3383995130135,17.1821008109519,
-13.9239031676938));
#104881=CARTESIAN_POINT('Ctrl Pts',(-19.3255888907522,17.1783270879104,
-13.9231050989033));
#104882=CARTESIAN_POINT('Ctrl Pts',(-19.3189624097634,17.1764102221578,
-13.9226939391777));
#104883=CARTESIAN_POINT('Ctrl Pts',(-19.301929102279,17.1715730310412,-13.9216412294542));
#104884=CARTESIAN_POINT('Ctrl Pts',(-19.2915089843051,17.1686999324512,
-13.9210012207575));
#104885=CARTESIAN_POINT('Ctrl Pts',(-19.2479272724313,17.1570417239593,
-13.9183405566925));
#104886=CARTESIAN_POINT('Ctrl Pts',(-19.2145755213211,17.1489832187947,
-13.9163434300315));
#104887=CARTESIAN_POINT('Ctrl Pts',(-19.1271788443181,17.1301021281015,
-13.9111993570371));
#104888=CARTESIAN_POINT('Ctrl Pts',(-19.0728802628434,17.1205726825023,
-13.9080917996022));
#104889=CARTESIAN_POINT('Ctrl Pts',(-18.9099124733886,17.098489543352,-13.8989473917473));
#104890=CARTESIAN_POINT('Ctrl Pts',(-18.8005786658719,17.092223515184,-13.8930592707198));
#104891=CARTESIAN_POINT('Ctrl Pts',(-18.6455299772278,17.0953551150471,
-13.8846160489244));
#104892=CARTESIAN_POINT('Ctrl Pts',(-18.5998525756087,17.0977597260572,
-13.8821156305693));
#104893=CARTESIAN_POINT('Ctrl Pts',(-18.5315820550036,17.1035761262075,
-13.8783162737223));
#104894=CARTESIAN_POINT('Ctrl Pts',(-18.5089070656659,17.1058773129884,
-13.8770439999209));
#104895=CARTESIAN_POINT('Ctrl Pts',(-18.485247947572,17.1086649923696,-13.8757017357188));
#104896=CARTESIAN_POINT('Ctrl Pts',(-18.484221746921,17.1087866682521,-13.8756434866502));
#104897=CARTESIAN_POINT('Ctrl Pts',(-18.4649615763543,17.1110846349086,
-13.8745496898693));
#104898=CARTESIAN_POINT('Ctrl Pts',(-18.4467570686057,17.113497276096,-13.8735065358503));
#104899=CARTESIAN_POINT('Ctrl Pts',(-18.3954595014673,17.1209760597273,
-13.870535093925));
#104900=CARTESIAN_POINT('Ctrl Pts',(-18.3624535443507,17.1265905657932,
-13.8685854768916));
#104901=CARTESIAN_POINT('Ctrl Pts',(-18.3227963977621,17.134308257534,-13.8661823321725));
#104902=CARTESIAN_POINT('Ctrl Pts',(-18.3160027248365,17.1356650220548,
-13.865768486132));
#104903=CARTESIAN_POINT('Ctrl Pts',(-18.3048595476132,17.1379473604288,
-13.8650859480077));
#104904=CARTESIAN_POINT('Ctrl Pts',(-18.3005060229945,17.1388533484867,
-13.8648183489069));
#104905=CARTESIAN_POINT('Ctrl Pts',(-18.2926706296167,17.1405097021833,
-13.8643349850882));
#104906=CARTESIAN_POINT('Ctrl Pts',(-18.2891877760491,17.1412551433535,
-13.8641195041359));
#104907=CARTESIAN_POINT('Ctrl Pts',(-18.281593592813,17.1429005934615,-13.8636482859043));
#104908=CARTESIAN_POINT('Ctrl Pts',(-18.2774831116099,17.1438040628687,
-13.8633923569547));
#104909=CARTESIAN_POINT('Ctrl Pts',(-18.2658662574508,17.1463937449515,
-13.8626666425523));
#104910=CARTESIAN_POINT('Ctrl Pts',(-18.2583664340568,17.1481086077841,
-13.8621952613406));
#104911=CARTESIAN_POINT('Ctrl Pts',(-18.2119004766103,17.1590000823457,
-13.8592577122704));
#104912=CARTESIAN_POINT('Ctrl Pts',(-18.1731944931754,17.1692389272465,
-13.856736303602));
#104913=CARTESIAN_POINT('Ctrl Pts',(-17.9690531403683,17.2294824916377,
-13.843121949756));
#104914=CARTESIAN_POINT('Ctrl Pts',(-17.8099143250524,17.2985080203104,
-13.8314565276146));
#104915=CARTESIAN_POINT('Ctrl Pts',(-17.5755719392057,17.4363059996227,
-13.8138298892532));
#104916=CARTESIAN_POINT('Ctrl Pts',(-17.4938310886263,17.4924307398264,
-13.807566759031));
#104917=CARTESIAN_POINT('Ctrl Pts',(-17.4053921742042,17.5627631149222,
-13.8006702907172));
#104918=CARTESIAN_POINT('Ctrl Pts',(-17.3945602821391,17.5715534955558,
-13.7998232416422));
#104919=CARTESIAN_POINT('Ctrl Pts',(-17.3773802816722,17.5857794750148,
-13.7984757295764));
#104920=CARTESIAN_POINT('Ctrl Pts',(-17.3709762400321,17.5911465967939,
-13.7979725135282));
#104921=CARTESIAN_POINT('Ctrl Pts',(-17.359692170942,17.6007178892845,-13.7970841427596));
#104922=CARTESIAN_POINT('Ctrl Pts',(-17.3547992702955,17.6049066547349,
-13.7966983642457));
#104923=CARTESIAN_POINT('Ctrl Pts',(-17.3446742698157,17.6136549597503,
-13.7958988340944));
#104924=CARTESIAN_POINT('Ctrl Pts',(-17.3394453146628,17.6182180332734,
-13.7954852352326));
#104925=CARTESIAN_POINT('Ctrl Pts',(-17.3259874393489,17.6300791915124,
-13.7944188904457));
#104926=CARTESIAN_POINT('Ctrl Pts',(-17.3177927204877,17.6374158992849,
-13.7937677649064));
#104927=CARTESIAN_POINT('Ctrl Pts',(-17.2830234651263,17.6690363268499,
-13.7909968280477));
#104928=CARTESIAN_POINT('Ctrl Pts',(-17.2570125373051,17.6939327189636,
-13.7889031074881));
#104929=CARTESIAN_POINT('Ctrl Pts',(-17.1901468282785,17.7612841007466,
-13.7834508714955));
#104930=CARTESIAN_POINT('Ctrl Pts',(-17.1504065275373,17.8048025452666,
-13.7801382302178));
#104931=CARTESIAN_POINT('Ctrl Pts',(-17.0043329347156,17.9788221669772,
-13.7675424840969));
#104932=CARTESIAN_POINT('Ctrl Pts',(-16.91190054555,18.1201487556587,-13.7586861849334));
#104933=CARTESIAN_POINT('Ctrl Pts',(-16.8128696027153,18.3199647629898,
-13.7461588532331));
#104934=CARTESIAN_POINT('Ctrl Pts',(-16.7904740252312,18.369934313279,-13.7430207505521));
#104935=CARTESIAN_POINT('Ctrl Pts',(-16.7667664136729,18.4288503968053,
-13.7392524561609));
#104936=CARTESIAN_POINT('Ctrl Pts',(-16.7635416844412,18.4370103323876,
-13.7387290500662));
#104937=CARTESIAN_POINT('Ctrl Pts',(-16.7587418676888,18.4493803350026,
-13.7379330031894));
#104938=CARTESIAN_POINT('Ctrl Pts',(-16.7571292660949,18.4535758757834,
-13.7376625586426));
#104939=CARTESIAN_POINT('Ctrl Pts',(-16.7542617223017,18.4611079682206,
-13.7371761819725));
#104940=CARTESIAN_POINT('Ctrl Pts',(-16.753001835874,18.4644425802715,-13.7369605498521));
#104941=CARTESIAN_POINT('Ctrl Pts',(-16.7502860217403,18.4716859597222,
-13.7364914883805));
#104942=CARTESIAN_POINT('Ctrl Pts',(-16.7488332412056,18.4755958004064,
-13.7362378809895));
#104943=CARTESIAN_POINT('Ctrl Pts',(-16.7447936058274,18.4865667916328,
-13.7355251449198));
#104944=CARTESIAN_POINT('Ctrl Pts',(-16.7422328372145,18.4936373878204,
-13.7350645082201));
#104945=CARTESIAN_POINT('Ctrl Pts',(-16.7273185026433,18.5355132218763,
-13.732329386372));
#104946=CARTESIAN_POINT('Ctrl Pts',(-16.7158405901155,18.5706210247756,
-13.7300079385062));
#104947=CARTESIAN_POINT('Ctrl Pts',(-16.6814134294518,18.686065294998,-13.7223225020622));
#104948=CARTESIAN_POINT('Ctrl Pts',(-16.6623005532234,18.7674600858583,
-13.7168258124974));
#104949=CARTESIAN_POINT('Ctrl Pts',(-16.6172530614757,19.0275869716926,
-13.6993884806524));
#104950=CARTESIAN_POINT('Ctrl Pts',(-16.6093169881871,19.2086559989151,
-13.6875186961139));
#104951=CARTESIAN_POINT('Ctrl Pts',(-16.6263536592911,19.4110650139397,
-13.675020974006));
#104952=CARTESIAN_POINT('Ctrl Pts',(-16.628608071998,19.4335398814456,-13.673642563196));
#104953=CARTESIAN_POINT('Ctrl Pts',(-16.6323187098712,19.4653906668255,
-13.6717016683274));
#104954=CARTESIAN_POINT('Ctrl Pts',(-16.6334788743084,19.4747989039789,
-13.6711299140231));
#104955=CARTESIAN_POINT('Ctrl Pts',(-16.635470666768,19.4901040960875,-13.6702022466815));
#104956=CARTESIAN_POINT('Ctrl Pts',(-16.6362640432706,19.4960058172362,
-13.6698451310404));
#104957=CARTESIAN_POINT('Ctrl Pts',(-16.6379803606692,19.5083775079965,
-13.6690977341825));
#104958=CARTESIAN_POINT('Ctrl Pts',(-16.6389083829206,19.5148467183352,
-13.6687076178036));
#104959=CARTESIAN_POINT('Ctrl Pts',(-16.641194218732,19.5302726512531,-13.6677790026042));
#104960=CARTESIAN_POINT('Ctrl Pts',(-16.6425796019414,19.5392252068562,
-13.6672413821677));
#104961=CARTESIAN_POINT('Ctrl Pts',(-16.647475947128,19.5695757453257,-13.6654230010135));
#104962=CARTESIAN_POINT('Ctrl Pts',(-16.6512582543336,19.5909290204605,
-13.6641508429832));
#104963=CARTESIAN_POINT('Ctrl Pts',(-16.6739143739679,19.7083050591278,
-13.6571919846735));
#104964=CARTESIAN_POINT('Ctrl Pts',(-16.6991014204847,19.8029933598678,
-13.6517118025733));
#104965=CARTESIAN_POINT('Ctrl Pts',(-16.7845100294689,20.0529092843735,
-13.6372003899247));
#104966=CARTESIAN_POINT('Ctrl Pts',(-16.8566009285505,20.2033124793429,
-13.6284399588336));
#104967=CARTESIAN_POINT('Ctrl Pts',(-16.965822299614,20.3757640498268,-13.6167945096372));
#104968=CARTESIAN_POINT('Ctrl Pts',(-16.9869731290592,20.4072543143438,
-13.6145932087564));
#104969=CARTESIAN_POINT('Ctrl Pts',(-17.0131367931583,20.4440331797615,
-13.6119102370081));
#104970=CARTESIAN_POINT('Ctrl Pts',(-17.0173467283316,20.4498876222483,
-13.6114796956935));
#104971=CARTESIAN_POINT('Ctrl Pts',(-17.0242519025832,20.4593873578055,
-13.6107752057976));
#104972=CARTESIAN_POINT('Ctrl Pts',(-17.0269291255608,20.4630457581544,
-13.6105024729501));
#104973=CARTESIAN_POINT('Ctrl Pts',(-17.0317342109016,20.4695678017357,
-13.610013639717));
#104974=CARTESIAN_POINT('Ctrl Pts',(-17.0338575797378,20.4724346906857,
-13.6097978523477));
#104975=CARTESIAN_POINT('Ctrl Pts',(-17.0384623229055,20.478619086361,-13.6093303728619));
#104976=CARTESIAN_POINT('Ctrl Pts',(-17.0409461565695,20.4819346344795,
-13.609078513066));
#104977=CARTESIAN_POINT('Ctrl Pts',(-17.0478880593633,20.4911445786532,
-13.6083754951136));
#104978=CARTESIAN_POINT('Ctrl Pts',(-17.0523672361996,20.4970228857299,
-13.6079228931589));
#104979=CARTESIAN_POINT('Ctrl Pts',(-17.0781160324881,20.5304501241866,
-13.605327403509));
#104980=CARTESIAN_POINT('Ctrl Pts',(-17.1000303869053,20.55749297156,-13.6031428598908));
#104981=CARTESIAN_POINT('Ctrl Pts',(-17.1716866032175,20.6415923157882,
-13.5961074696339));
#104982=CARTESIAN_POINT('Ctrl Pts',(-17.2238244848166,20.6965254523574,
-13.5911459833851));
#104983=CARTESIAN_POINT('Ctrl Pts',(-17.4185998537363,20.8808709963673,
-13.5734542658346));
#104984=CARTESIAN_POINT('Ctrl Pts',(-17.5758436885065,20.993540735882,-13.5607397498693));
#104985=CARTESIAN_POINT('Ctrl Pts',(-17.7650385167635,21.0933542291536,
-13.5475951513949));
#104986=CARTESIAN_POINT('Ctrl Pts',(-17.7840503645629,21.1030199635231,
-13.5462947035357));
#104987=CARTESIAN_POINT('Ctrl Pts',(-17.81068968032,21.1160607570359,-13.5445001456819));
#104988=CARTESIAN_POINT('Ctrl Pts',(-17.8181954248019,21.1196802816547,
-13.5439975280646));
#104989=CARTESIAN_POINT('Ctrl Pts',(-17.8311827020417,21.1258489411309,
-13.5431329578895));
#104990=CARTESIAN_POINT('Ctrl Pts',(-17.836654101312,21.1284190674262,-13.5427702793366));
#104991=CARTESIAN_POINT('Ctrl Pts',(-17.8480021265544,21.1336904582237,
-13.5420212440518));
#104992=CARTESIAN_POINT('Ctrl Pts',(-17.8538802796671,21.136388300891,-13.5416350086013));
#104993=CARTESIAN_POINT('Ctrl Pts',(-17.8676672067033,21.1426396311931,
-13.5407331680261));
#104994=CARTESIAN_POINT('Ctrl Pts',(-17.8755856676788,21.1461715714667,
-13.5402183079099));
#104995=CARTESIAN_POINT('Ctrl Pts',(-17.901332332674,21.1574664533431,-13.5385541310275));
#104996=CARTESIAN_POINT('Ctrl Pts',(-17.9192461697134,21.1650325819966,
-13.537411530066));
#104997=CARTESIAN_POINT('Ctrl Pts',(-18.0112101433606,21.2023900855222,
-13.5316196923666));
#104998=CARTESIAN_POINT('Ctrl Pts',(-18.0868022542763,21.2282250056676,
-13.527104866799));
#104999=CARTESIAN_POINT('Ctrl Pts',(-18.3235024776175,21.2944401897104,
-13.5134723877485));
#105000=CARTESIAN_POINT('Ctrl Pts',(-18.4880137295316,21.3201978023287,
-13.5047300554365));
#105001=CARTESIAN_POINT('Ctrl Pts',(-18.7116111523022,21.3286710825945,
-13.4921915777757));
#105002=CARTESIAN_POINT('Ctrl Pts',(-18.7694491256858,21.3284924244502,
-13.4888843237578));
#105003=CARTESIAN_POINT('Ctrl Pts',(-18.8360826012219,21.3255560220886,
-13.4849275967332));
#105004=CARTESIAN_POINT('Ctrl Pts',(-18.844961023476,21.3251087183569,-13.4843973792927));
#105005=CARTESIAN_POINT('Ctrl Pts',(-18.8583485193683,21.3243496805579,
-13.4835929834094));
#105006=CARTESIAN_POINT('Ctrl Pts',(-18.8628599713676,21.3240793959273,
-13.4833210704686));
#105007=CARTESIAN_POINT('Ctrl Pts',(-18.8709299673567,21.3235699762403,
-13.4828331206923));
#105008=CARTESIAN_POINT('Ctrl Pts',(-18.8744888027043,21.3233362934241,
-13.482617392214));
#105009=CARTESIAN_POINT('Ctrl Pts',(-18.8821901688445,21.3228110518978,
-13.4821493606945));
#105010=CARTESIAN_POINT('Ctrl Pts',(-18.8863323802574,21.322516301216,-13.4818968863199));
#105011=CARTESIAN_POINT('Ctrl Pts',(-18.8978892799454,21.321659754074,-13.4811904555982));
#105012=CARTESIAN_POINT('Ctrl Pts',(-18.9053018304987,21.3210710823677,
-13.4807350330425));
#105013=CARTESIAN_POINT('Ctrl Pts',(-18.9481185441162,21.3174436715999,
-13.4780915854121));
#105014=CARTESIAN_POINT('Ctrl Pts',(-18.9834426064714,21.3135531465626,
-13.4758601188409));
#105015=CARTESIAN_POINT('Ctrl Pts',(-19.096255821416,21.2982453979133,-13.4686060143291));
#105016=CARTESIAN_POINT('Ctrl Pts',(-19.1732129525762,21.2834171772923,
-13.4634655010647));
#105017=CARTESIAN_POINT('Ctrl Pts',(-19.4318699454908,21.2185229676173,
-13.4458644097813));
#105018=CARTESIAN_POINT('Ctrl Pts',(-19.607682314076,21.1484929743937,-13.4334408226361));
#105019=CARTESIAN_POINT('Ctrl Pts',(-19.7909251529856,21.0454136871527,
-13.4205151030088));
#105020=CARTESIAN_POINT('Ctrl Pts',(-19.8097618252229,21.0344310806344,
-13.4191851636067));
#105021=CARTESIAN_POINT('Ctrl Pts',(-19.8362649764433,21.0184249039051,
-13.4173115756307));
#105022=CARTESIAN_POINT('Ctrl Pts',(-19.8440732020395,21.0136398286361,
-13.4167592887449));
#105023=CARTESIAN_POINT('Ctrl Pts',(-19.857337529036,21.0053922501973,-13.4158204933659));
#105024=CARTESIAN_POINT('Ctrl Pts',(-19.8628092252545,21.0019551881963,
-13.41543305558));
#105025=CARTESIAN_POINT('Ctrl Pts',(-19.8737393797323,20.9950193889556,
-13.4146587325803));
#105026=CARTESIAN_POINT('Ctrl Pts',(-19.8791976724626,20.9915205211706,
-13.4142718577985));
#105027=CARTESIAN_POINT('Ctrl Pts',(-19.8901575575369,20.9844237824799,
-13.4134946063724));
#105028=CARTESIAN_POINT('Ctrl Pts',(-19.8956586381718,20.9808252512499,
-13.4131042599969));
#105029=CARTESIAN_POINT('Ctrl Pts',(-19.9156418476291,20.9676199254016,
-13.4116853938145));
#105030=CARTESIAN_POINT('Ctrl Pts',(-19.930022557703,20.9578603512038,-13.4106626064586));
#105031=CARTESIAN_POINT('Ctrl Pts',(-19.9629011623044,20.9349506769682,
-13.4083190648746));
#105032=CARTESIAN_POINT('Ctrl Pts',(-19.9813111987015,20.9216778869677,
-13.4070029965833));
#105033=CARTESIAN_POINT('Ctrl Pts',(-20.043425193603,20.8753606191372,-13.4025447853776));
#105034=CARTESIAN_POINT('Ctrl Pts',(-20.0860597034314,20.8409158881622,
-13.3994544338268));
#105035=CARTESIAN_POINT('Ctrl Pts',(-20.2094383406355,20.7330609753651,
-13.3903400574244));
#105036=CARTESIAN_POINT('Ctrl Pts',(-20.2858949755795,20.6550259029552,
-13.3844648581662));
#105037=CARTESIAN_POINT('Ctrl Pts',(-20.4326298357147,20.48008075314,-13.3720352395967));
#105038=CARTESIAN_POINT('Ctrl Pts',(-20.5013951255844,20.3824160193898,
-13.3654876689711));
#105039=CARTESIAN_POINT('Ctrl Pts',(-20.5663658998535,20.2712898997211,
-13.3578588092128));
#105040=CARTESIAN_POINT('Ctrl Pts',(-20.5711109271987,20.2630470027188,
-13.3572918904577));
#105041=CARTESIAN_POINT('Ctrl Pts',(-20.5780600881861,20.2507847859239,
-13.3564465772265));
#105042=CARTESIAN_POINT('Ctrl Pts',(-20.5803070459711,20.246789699201,-13.3561708643815));
#105043=CARTESIAN_POINT('Ctrl Pts',(-20.5842819781142,20.2396682466034,
-13.3556787914355));
#105044=CARTESIAN_POINT('Ctrl Pts',(-20.5860150316978,20.2365447733964,
-13.3554627612576));
#105045=CARTESIAN_POINT('Ctrl Pts',(-20.5897243136761,20.2298194882414,
-13.3549971575745));
#105046=CARTESIAN_POINT('Ctrl Pts',(-20.59169793634,20.2262163585386,-13.3547474291575));
#105047=CARTESIAN_POINT('Ctrl Pts',(-20.5971174093858,20.2162536185894,
-13.3540562087744));
#105048=CARTESIAN_POINT('Ctrl Pts',(-20.6005411355865,20.2098821274447,
-13.3536133492945));
#105049=CARTESIAN_POINT('Ctrl Pts',(-20.6191285946934,20.1748619561541,
-13.3511753636231));
#105050=CARTESIAN_POINT('Ctrl Pts',(-20.6336645794219,20.1458871099919,
-13.3491441730077));
#105051=CARTESIAN_POINT('Ctrl Pts',(-20.7171728107169,19.9694330184984,
-13.3367407938375));
#105052=CARTESIAN_POINT('Ctrl Pts',(-20.7696074828148,19.8147359774947,
-13.3257767183171));
#105053=CARTESIAN_POINT('Ctrl Pts',(-20.8169122812128,19.5944926868546,
-13.3110623029466));
#105054=CARTESIAN_POINT('Ctrl Pts',(-20.8273203164416,19.5328715338825,
-13.3070312374439));
#105055=CARTESIAN_POINT('Ctrl Pts',(-20.838240896145,19.4445832687708,-13.3013963914024));
#105056=CARTESIAN_POINT('Ctrl Pts',(-20.8409993766864,19.4182308218197,
-13.2997319479751));
#105057=CARTESIAN_POINT('Ctrl Pts',(-20.8463154919444,19.3562227468594,
-13.2958566623018));
#105058=CARTESIAN_POINT('Ctrl Pts',(-20.8484662878358,19.3205396989405,
-13.2936585268251));
#105059=CARTESIAN_POINT('Ctrl Pts',(-20.8501018463093,19.2736623165284,
-13.2908109024725));
#105060=CARTESIAN_POINT('Ctrl Pts',(-20.8504028278496,19.2625040543427,
-13.2901360432393));
#105061=CARTESIAN_POINT('Ctrl Pts',(-20.8507477574777,19.2444074923976,
-13.2890462302954));
#105062=CARTESIAN_POINT('Ctrl Pts',(-20.8508458708876,19.237470550147,-13.2886295872446));
#105063=CARTESIAN_POINT('Ctrl Pts',(-20.8509497984026,19.2262074011857,
-13.2879548791866));
#105064=CARTESIAN_POINT('Ctrl Pts',(-20.8509764542477,19.2218814795907,
-13.287696163653));
#105065=CARTESIAN_POINT('Ctrl Pts',(-20.8509965706155,19.2153852145476,
-13.287308277758));
#105066=CARTESIAN_POINT('Ctrl Pts',(-20.8509999537594,19.2132149334439,
-13.2871787977096));
#105067=CARTESIAN_POINT('Ctrl Pts',(-20.8509999995292,19.2110446460074,
-13.2870494219157));
#105068=CARTESIAN_POINT('Ctrl Pts',(-20.8509999986719,19.2109250126718,
-13.2890562789747));
#105069=CARTESIAN_POINT('Ctrl Pts',(-20.8509972774554,19.1341011600837,
-13.2844612169106));
#105070=CARTESIAN_POINT('Ctrl Pts',(-20.8468084619602,19.0573628290618,
-13.2798661548465));
#105071=CARTESIAN_POINT('Ctrl Pts',(-20.8384871131119,18.9811674723936,
-13.2752710927824));
#105072=CARTESIAN_POINT('Ctrl Pts',(-20.8301538008465,18.9048625713658,
-13.2706694245004));
#105073=CARTESIAN_POINT('Ctrl Pts',(-20.8176761741998,18.8291026018815,
-13.2660677562184));
#105074=CARTESIAN_POINT('Ctrl Pts',(-20.8011589270513,18.7543349473497,
-13.2614660879363));
#105075=CARTESIAN_POINT('Ctrl Pts',(-20.7846027399158,18.679391025461,-13.2568535710606));
#105076=CARTESIAN_POINT('Ctrl Pts',(-20.763988012731,18.6054444843118,-13.2522410541849));
#105077=CARTESIAN_POINT('Ctrl Pts',(-20.7394693419458,18.5329279400275,
-13.2476285373092));
#105078=CARTESIAN_POINT('Ctrl Pts',(-20.734030977206,18.5168434050645,-13.2466054578218));
#105079=CARTESIAN_POINT('Ctrl Pts',(-20.7284007341625,18.5008291398821,
-13.2455823783344));
#105080=CARTESIAN_POINT('Ctrl Pts',(-20.7225806137986,18.4848897174502,
-13.2445592988469));
#105081=CARTESIAN_POINT('Origin',(-18.734,19.211,0.));
#105082=CARTESIAN_POINT('',(-20.7242505411024,18.4842642021379,-12.4443820858314));
#105083=CARTESIAN_POINT('',(-20.7225805288028,18.4848894846743,-12.6679318969538));
#105084=CARTESIAN_POINT('',(-20.7225806137986,18.4848897174502,0.));
#105085=CARTESIAN_POINT('Ctrl Pts',(-20.7225805288028,18.4848894846743,
-12.6679318969538));
#105086=CARTESIAN_POINT('Ctrl Pts',(-20.7627961214462,18.5950269125135,
-12.6745735586325));
#105087=CARTESIAN_POINT('Ctrl Pts',(-20.7938157091376,18.7083782681631,
-12.6809438446479));
#105088=CARTESIAN_POINT('Ctrl Pts',(-20.8390879891312,18.9517192360552,
-12.6943852386175));
#105089=CARTESIAN_POINT('Ctrl Pts',(-20.8510398088253,19.0815565850429,
-12.7014276439781));
#105090=CARTESIAN_POINT('Ctrl Pts',(-20.8509988957047,19.2149244778125,
-12.7092186304204));
#105091=CARTESIAN_POINT('Ctrl Pts',(-20.8509902911661,19.218199498468,-12.7094102988555));
#105092=CARTESIAN_POINT('Ctrl Pts',(-20.8508966099817,19.2371332231321,
-12.7105204774892));
#105093=CARTESIAN_POINT('Ctrl Pts',(-20.8506454015414,19.2527901243868,
-12.7114468030206));
#105094=CARTESIAN_POINT('Ctrl Pts',(-20.8500635586938,19.2742256918366,
-12.7127281078718));
#105095=CARTESIAN_POINT('Ctrl Pts',(-20.849882869319,19.2800083623479,-12.7130750707398));
#105096=CARTESIAN_POINT('Ctrl Pts',(-20.8495580050343,19.2891981881347,
-12.7136286418556));
#105097=CARTESIAN_POINT('Ctrl Pts',(-20.8494292955161,19.292605910229,-12.713834390178));
#105098=CARTESIAN_POINT('Ctrl Pts',(-20.8491463964198,19.2996449787777,
-12.7142603993217));
#105099=CARTESIAN_POINT('Ctrl Pts',(-20.8489910889964,19.303276233328,-12.7144807243681));
#105100=CARTESIAN_POINT('Ctrl Pts',(-20.8485986103281,19.311930701008,-12.7150071394247));
#105101=CARTESIAN_POINT('Ctrl Pts',(-20.8483528906747,19.3169534884063,
-12.7153137043087));
#105102=CARTESIAN_POINT('Ctrl Pts',(-20.8474631220289,19.3339036609023,
-12.7163516895652));
#105103=CARTESIAN_POINT('Ctrl Pts',(-20.8467360360084,19.345826203305,-12.7170875375017));
#105104=CARTESIAN_POINT('Ctrl Pts',(-20.8368854509554,19.4875959922649,
-12.7259006911209));
#105105=CARTESIAN_POINT('Ctrl Pts',(-20.8159065091064,19.6163281873859,
-12.7345181394112));
#105106=CARTESIAN_POINT('Ctrl Pts',(-20.7425052049445,19.8994378314436,
-12.7538447946671));
#105107=CARTESIAN_POINT('Ctrl Pts',(-20.6838198863416,20.0513933538053,
-12.7644508258067));
#105108=CARTESIAN_POINT('Ctrl Pts',(-20.5973016052834,20.2161660124741,
-12.7759141602397));
#105109=CARTESIAN_POINT('Ctrl Pts',(-20.5859225279541,20.2369798278505,
-12.7773627919499));
#105110=CARTESIAN_POINT('Ctrl Pts',(-20.5694165603161,20.2660016587093,
-12.7793842980244));
#105111=CARTESIAN_POINT('Ctrl Pts',(-20.5645798741583,20.2743718911735,
-12.7799675185626));
#105112=CARTESIAN_POINT('Ctrl Pts',(-20.5566541592534,20.287873568392,-12.7809086898092));
#105113=CARTESIAN_POINT('Ctrl Pts',(-20.5536004316783,20.2930254787789,
-12.7812679136698));
#105114=CARTESIAN_POINT('Ctrl Pts',(-20.5471836319514,20.3037472023617,
-12.7820157309393));
#105115=CARTESIAN_POINT('Ctrl Pts',(-20.543816658123,20.3093146165302,-12.7824041769744));
#105116=CARTESIAN_POINT('Ctrl Pts',(-20.5357844682834,20.3224589063981,
-12.7833216308878));
#105117=CARTESIAN_POINT('Ctrl Pts',(-20.5310970210085,20.3300221050202,
-12.783849816171));
#105118=CARTESIAN_POINT('Ctrl Pts',(-20.5153276311569,20.3551113721179,
-12.7856031001709));
#105119=CARTESIAN_POINT('Ctrl Pts',(-20.5040356777052,20.3725045010785,
-12.7868204231206));
#105120=CARTESIAN_POINT('Ctrl Pts',(-20.442393710235,20.4644651884676,-12.7932713762075));
#105121=CARTESIAN_POINT('Ctrl Pts',(-20.3875813317937,20.535936038902,-12.7983320606583));
#105122=CARTESIAN_POINT('Ctrl Pts',(-20.2392359525445,20.7057627660624,
-12.8107690126813));
#105123=CARTESIAN_POINT('Ctrl Pts',(-20.1405024887274,20.7990174772575,
-12.8179812878458));
#105124=CARTESIAN_POINT('Ctrl Pts',(-19.9740205527178,20.9284755678176,
-12.8296571181667));
#105125=CARTESIAN_POINT('Ctrl Pts',(-19.912079634336,20.9715394382112,-12.8339176887515));
#105126=CARTESIAN_POINT('Ctrl Pts',(-19.839912426887,21.0161971525049,-12.8389475073708));
#105127=CARTESIAN_POINT('Ctrl Pts',(-19.8318094457829,21.0211363121381,
-12.8395131656306));
#105128=CARTESIAN_POINT('Ctrl Pts',(-19.8197474895229,21.0283778804483,
-12.8403569549728));
#105129=CARTESIAN_POINT('Ctrl Pts',(-19.8158136803405,21.0307222676749,
-12.8406324184359));
#105130=CARTESIAN_POINT('Ctrl Pts',(-19.8087982317679,21.0348723963692,
-12.8411242186081));
#105131=CARTESIAN_POINT('Ctrl Pts',(-19.8057195989282,21.0366831209964,
-12.8413402268077));
#105132=CARTESIAN_POINT('Ctrl Pts',(-19.7990874991308,21.0405612917087,
-12.8418059799307));
#105133=CARTESIAN_POINT('Ctrl Pts',(-19.7955326400418,21.0426261502789,
-12.842055880805));
#105134=CARTESIAN_POINT('Ctrl Pts',(-19.7856956750312,21.0483017470527,
-12.8427480536842));
#105135=CARTESIAN_POINT('Ctrl Pts',(-19.7794010801632,21.0518905672797,
-12.8431916992939));
#105136=CARTESIAN_POINT('Ctrl Pts',(-19.7446853690071,21.0714480227753,
-12.8456419493298));
#105137=CARTESIAN_POINT('Ctrl Pts',(-19.7159183900048,21.086789904366,-12.8476850385778));
#105138=CARTESIAN_POINT('Ctrl Pts',(-19.5415656814313,21.1746653762207,
-12.8600924188335));
#105139=CARTESIAN_POINT('Ctrl Pts',(-19.3883725996815,21.2308862539321,
-12.8710455923524));
#105140=CARTESIAN_POINT('Ctrl Pts',(-19.1167165575343,21.2963914460537,
-12.8892984491996));
#105141=CARTESIAN_POINT('Ctrl Pts',(-19.0010936239427,21.3143302748905,
-12.8967380038184));
#105142=CARTESIAN_POINT('Ctrl Pts',(-18.8703108366637,21.3236553277636,
-12.904743864424));
#105143=CARTESIAN_POINT('Ctrl Pts',(-18.8560477411838,21.3245272751275,
-12.9056118247965));
#105144=CARTESIAN_POINT('Ctrl Pts',(-18.8333331545337,21.325685177977,-12.90698611335));
#105145=CARTESIAN_POINT('Ctrl Pts',(-18.8248870821312,21.3260650153331,
-12.907495369466));
#105146=CARTESIAN_POINT('Ctrl Pts',(-18.8099870549081,21.3266456831299,
-12.9083907423932));
#105147=CARTESIAN_POINT('Ctrl Pts',(-18.8035340746435,21.3268676005261,
-12.9087775153074));
#105148=CARTESIAN_POINT('Ctrl Pts',(-18.7901850990114,21.3272655358598,
-12.9095755850914));
#105149=CARTESIAN_POINT('Ctrl Pts',(-18.7832890487378,21.327437378007,-12.9099867465678));
#105150=CARTESIAN_POINT('Ctrl Pts',(-18.7655855976869,21.3277919548024,
-12.9110394661193));
#105151=CARTESIAN_POINT('Ctrl Pts',(-18.7547773300265,21.3279256337938,
-12.9116794828368));
#105152=CARTESIAN_POINT('Ctrl Pts',(-18.7096624265858,21.3281380695596,
-12.9143402249152));
#105153=CARTESIAN_POINT('Ctrl Pts',(-18.6753563225963,21.3274656951576,
-12.9163374198074));
#105154=CARTESIAN_POINT('Ctrl Pts',(-18.5860257135005,21.3235409957281,
-12.9214817082814));
#105155=CARTESIAN_POINT('Ctrl Pts',(-18.5310841572953,21.3189733523813,
-12.9245894086367));
#105156=CARTESIAN_POINT('Ctrl Pts',(-18.3678444128874,21.2989598160033,
-12.9337340658193));
#105157=CARTESIAN_POINT('Ctrl Pts',(-18.2604996768575,21.2772633991256,
-12.9396222940831));
#105158=CARTESIAN_POINT('Ctrl Pts',(-18.1111192258013,21.2348130471402,
-12.9480772179085));
#105159=CARTESIAN_POINT('Ctrl Pts',(-18.0673482912213,21.220819635332,-12.9505893087198));
#105160=CARTESIAN_POINT('Ctrl Pts',(-18.0030685432172,21.197938622132,-12.954373240686));
#105161=CARTESIAN_POINT('Ctrl Pts',(-17.9821883216845,21.1901323943882,
-12.9556176305286));
#105162=CARTESIAN_POINT('Ctrl Pts',(-17.9135820707828,21.1632410778597,
-12.9597685686341));
#105163=CARTESIAN_POINT('Ctrl Pts',(-17.8664314071896,21.1427491089816,
-12.9627219879601));
#105164=CARTESIAN_POINT('Ctrl Pts',(-17.8129719811901,21.1171632770823,
-12.9662396476612));
#105165=CARTESIAN_POINT('Ctrl Pts',(-17.8058857934373,21.1137230659092,
-12.9667094290941));
#105166=CARTESIAN_POINT('Ctrl Pts',(-17.7946183712581,21.1081750261986,
-12.9674622714523));
#105167=CARTESIAN_POINT('Ctrl Pts',(-17.7904245675576,21.1060926960909,
-12.9677437872589));
#105168=CARTESIAN_POINT('Ctrl Pts',(-17.7830248567056,21.1023878996941,
-12.9682428720952));
#105169=CARTESIAN_POINT('Ctrl Pts',(-17.7798161289571,21.1007711634908,
-12.9684600812003));
#105170=CARTESIAN_POINT('Ctrl Pts',(-17.7730410488711,21.0973358449092,
-12.9689204059536));
#105171=CARTESIAN_POINT('Ctrl Pts',(-17.7694757900858,21.0955153417838,
-12.969163636482));
#105172=CARTESIAN_POINT('Ctrl Pts',(-17.7599052790968,21.0905941456448,
-12.9698191897808));
#105173=CARTESIAN_POINT('Ctrl Pts',(-17.7539097354699,21.0874748194837,
-12.9702326604402));
#105174=CARTESIAN_POINT('Ctrl Pts',(-17.7247052097881,21.0721023148026,
-12.9722599812006));
#105175=CARTESIAN_POINT('Ctrl Pts',(-17.7017116378027,21.0594475622684,
-12.9738972755162));
#105176=CARTESIAN_POINT('Ctrl Pts',(-17.6365240884844,21.0219753017653,
-12.9786453038926));
#105177=CARTESIAN_POINT('Ctrl Pts',(-17.5949491518425,20.9961183301519,
-12.9818036102215));
#105178=CARTESIAN_POINT('Ctrl Pts',(-17.4740587952986,20.9149888710586,
-12.9913040435502));
#105179=CARTESIAN_POINT('Ctrl Pts',(-17.3975903533404,20.855700267134,-12.9977329730545));
#105180=CARTESIAN_POINT('Ctrl Pts',(-17.2201680483101,20.697569037905,-13.013368531114));
#105181=CARTESIAN_POINT('Ctrl Pts',(-17.1245175066716,20.5934449851206,
-13.0224360754053));
#105182=CARTESIAN_POINT('Ctrl Pts',(-17.0313564972683,20.46913277953,-13.0319214321291));
#105183=CARTESIAN_POINT('Ctrl Pts',(-17.0229070541902,20.4576169960404,
-13.0327889835561));
#105184=CARTESIAN_POINT('Ctrl Pts',(-17.0096436019779,20.439151235634,-13.0341627490327));
#105185=CARTESIAN_POINT('Ctrl Pts',(-17.004753675755,20.4322565653094,-13.0346718875507));
#105186=CARTESIAN_POINT('Ctrl Pts',(-16.9962016666346,20.4200441007411,
-13.0355671237013));
#105187=CARTESIAN_POINT('Ctrl Pts',(-16.9925223968725,20.4147385281789,
-13.0359538768059));
#105188=CARTESIAN_POINT('Ctrl Pts',(-16.9849620308511,20.4037291297265,
-13.0367519727492));
#105189=CARTESIAN_POINT('Ctrl Pts',(-16.9810844247459,20.3980229914313,
-13.037163179864));
#105190=CARTESIAN_POINT('Ctrl Pts',(-16.9712013907032,20.3833254539917,
-13.0382161550684));
#105191=CARTESIAN_POINT('Ctrl Pts',(-16.9652367807699,20.3743067471134,
-13.0388563803305));
#105192=CARTESIAN_POINT('Ctrl Pts',(-16.9406198273755,20.3364579564063,
-13.0415191501685));
#105193=CARTESIAN_POINT('Ctrl Pts',(-16.9226005855232,20.3072209693176,
-13.043518118474));
#105194=CARTESIAN_POINT('Ctrl Pts',(-16.8775016175344,20.2298950776539,
-13.0486680082594));
#105195=CARTESIAN_POINT('Ctrl Pts',(-16.8515761765729,20.1811621616415,
-13.0517794239177));
#105196=CARTESIAN_POINT('Ctrl Pts',(-16.7800136370308,20.032946388887,-13.0609305621458));
#105197=CARTESIAN_POINT('Ctrl Pts',(-16.74015199032,19.9308816318834,-13.0668215778965));
#105198=CARTESIAN_POINT('Ctrl Pts',(-16.6935657544593,19.777487575627,-13.0755499526949));
#105199=CARTESIAN_POINT('Ctrl Pts',(-16.6805355722498,19.728265481387,-13.0783345928624));
#105200=CARTESIAN_POINT('Ctrl Pts',(-16.6658182735494,19.6632838928989,
-13.0820414583301));
#105201=CARTESIAN_POINT('Ctrl Pts',(-16.6625152114379,19.647906313448,-13.0829209167307));
#105202=CARTESIAN_POINT('Ctrl Pts',(-16.6488821001186,19.5808033483538,
-13.0867737226768));
#105203=CARTESIAN_POINT('Ctrl Pts',(-16.6403167630758,19.5287431160823,
-13.0898016714684));
#105204=CARTESIAN_POINT('Ctrl Pts',(-16.632614976478,19.4677986341198,-13.0934472666022));
#105205=CARTESIAN_POINT('Ctrl Pts',(-16.6315783128438,19.4591684892992,
-13.0939658525503));
#105206=CARTESIAN_POINT('Ctrl Pts',(-16.6300882631347,19.4460839187503,
-13.0947559865968));
#105207=CARTESIAN_POINT('Ctrl Pts',(-16.6295957988882,19.4416339152661,
-13.0950253868715));
#105208=CARTESIAN_POINT('Ctrl Pts',(-16.6287367224732,19.4336392405892,
-13.095510652212));
#105209=CARTESIAN_POINT('Ctrl Pts',(-16.6283649410985,19.4300951792643,
-13.0957262232256));
#105210=CARTESIAN_POINT('Ctrl Pts',(-16.6275760431037,19.4223873790919,
-13.0961960507659));
#105211=CARTESIAN_POINT('Ctrl Pts',(-16.6271623281281,19.4182233913149,
-13.0964504902343));
#105212=CARTESIAN_POINT('Ctrl Pts',(-16.6260337072185,19.4065111162331,
-13.0971678686295));
#105213=CARTESIAN_POINT('Ctrl Pts',(-16.6253470121466,19.3989602641437,
-13.0976323467011));
#105214=CARTESIAN_POINT('Ctrl Pts',(-16.6214621588144,19.3535387328608,
-13.1004376574194));
#105215=CARTESIAN_POINT('Ctrl Pts',(-16.6192439488305,19.3155937351445,
-13.1028282446724));
#105216=CARTESIAN_POINT('Ctrl Pts',(-16.6152879465656,19.1899309489021,
-13.1108564482069));
#105217=CARTESIAN_POINT('Ctrl Pts',(-16.6179805452626,19.1021680075429,
-13.1166390515131));
#105218=CARTESIAN_POINT('Ctrl Pts',(-16.6422709220074,18.8411604074901,
-13.1339594037061));
#105219=CARTESIAN_POINT('Ctrl Pts',(-16.6798383629085,18.6701165724637,
-13.1454065499973));
#105220=CARTESIAN_POINT('Ctrl Pts',(-16.7456645979487,18.4838525846326,
-13.1575672194748));
#105221=CARTESIAN_POINT('Ctrl Pts',(-16.7537054574057,18.4622312604318,
-13.1589753793716));
#105222=CARTESIAN_POINT('Ctrl Pts',(-16.7655760968725,18.4318416712428,
-13.1609504102105));
#105223=CARTESIAN_POINT('Ctrl Pts',(-16.7691141661991,18.4229619117763,
-13.1615270009044));
#105224=CARTESIAN_POINT('Ctrl Pts',(-16.7749591997906,18.4085763136206,
-13.1624603584571));
#105225=CARTESIAN_POINT('Ctrl Pts',(-16.777229494256,18.4030558074147,-13.1628183575218));
#105226=CARTESIAN_POINT('Ctrl Pts',(-16.782029416633,18.3915231024568,-13.1635658960731));
#105227=CARTESIAN_POINT('Ctrl Pts',(-16.7845635461611,18.3855128360478,
-13.1639552782064));
#105228=CARTESIAN_POINT('Ctrl Pts',(-16.7906560120549,18.3712476872335,
-13.1648790412546));
#105229=CARTESIAN_POINT('Ctrl Pts',(-16.7942392456181,18.3630035248689,
-13.1654125680824));
#105230=CARTESIAN_POINT('Ctrl Pts',(-16.8064770418231,18.3353307669333,
-13.1672024943917));
#105231=CARTESIAN_POINT('Ctrl Pts',(-16.8153720255238,18.3160094390806,
-13.1684506581482));
#105232=CARTESIAN_POINT('Ctrl Pts',(-16.8912559679692,18.1575101867887,
-13.1786845740511));
#105233=CARTESIAN_POINT('Ctrl Pts',(-16.9730017473837,18.0259097224612,
-13.1871018353607));
#105234=CARTESIAN_POINT('Ctrl Pts',(-17.1527681058354,17.7967505041328,
-13.2029185394502));
#105235=CARTESIAN_POINT('Ctrl Pts',(-17.2474049029209,17.6975864496225,
-13.2103041823479));
#105236=CARTESIAN_POINT('Ctrl Pts',(-17.3627251652693,17.5980718354622,
-13.2192364398674));
#105237=CARTESIAN_POINT('Ctrl Pts',(-17.3746370899476,17.5880199067183,
-13.2201585438136));
#105238=CARTESIAN_POINT('Ctrl Pts',(-17.3911125781449,17.5744256150461,
-13.221434895136));
#105239=CARTESIAN_POINT('Ctrl Pts',(-17.3955815924742,17.5707687632893,
-13.2217812058135));
#105240=CARTESIAN_POINT('Ctrl Pts',(-17.4027118081886,17.5649828783026,
-13.2223339932691));
#105241=CARTESIAN_POINT('Ctrl Pts',(-17.4053633239805,17.5628418773269,
-13.2225396144794));
#105242=CARTESIAN_POINT('Ctrl Pts',(-17.4108544057981,17.5584298934262,
-13.2229655825414));
#105243=CARTESIAN_POINT('Ctrl Pts',(-17.4136946484201,17.5561598269292,
-13.2231859946132));
#105244=CARTESIAN_POINT('Ctrl Pts',(-17.4204832692697,17.5507626172451,
-13.2237129833849));
#105245=CARTESIAN_POINT('Ctrl Pts',(-17.4244369748889,17.5476422359986,
-13.2240200376908));
#105246=CARTESIAN_POINT('Ctrl Pts',(-17.4378411420571,17.5371406843449,
-13.2250613832602));
#105247=CARTESIAN_POINT('Ctrl Pts',(-17.4473429689936,17.5298258677562,
-13.2258001403894));
#105248=CARTESIAN_POINT('Ctrl Pts',(-17.5586203541307,17.4456568204853,
-13.2344534853721));
#105249=CARTESIAN_POINT('Ctrl Pts',(-17.6670681667437,17.3780778595741,
-13.2428870751563));
#105250=CARTESIAN_POINT('Ctrl Pts',(-17.9283053822837,17.2463655514479,
-13.2622208253673));
#105251=CARTESIAN_POINT('Ctrl Pts',(-18.0839003419188,17.1895345787758,
-13.2730160026197));
#105252=CARTESIAN_POINT('Ctrl Pts',(-18.2675081190578,17.1459015602301,
-13.2846391316875));
#105253=CARTESIAN_POINT('Ctrl Pts',(-18.2905648462791,17.1408281288342,
-13.2860807622327));
#105254=CARTESIAN_POINT('Ctrl Pts',(-18.3231583579266,17.1342257633574,
-13.2880942222899));
#105255=CARTESIAN_POINT('Ctrl Pts',(-18.3326274551369,17.1323749328234,
-13.2886762884125));
#105256=CARTESIAN_POINT('Ctrl Pts',(-18.3479909466912,17.1294808826901,
-13.2896160980607));
#105257=CARTESIAN_POINT('Ctrl Pts',(-18.3538776135144,17.1283978302616,
-13.289975107578));
#105258=CARTESIAN_POINT('Ctrl Pts',(-18.3661753404608,17.1261891244055,
-13.2907228696037));
#105259=CARTESIAN_POINT('Ctrl Pts',(-18.3725871659861,17.1250680423293,
-13.2911114730229));
#105260=CARTESIAN_POINT('Ctrl Pts',(-18.3877912144908,17.1224818832629,
-13.292029998264));
#105261=CARTESIAN_POINT('Ctrl Pts',(-18.3965877653347,17.1210427194072,
-13.2925590921504));
#105262=CARTESIAN_POINT('Ctrl Pts',(-18.4253806663287,17.1165185684773,
-13.2942834919966));
#105263=CARTESIAN_POINT('Ctrl Pts',(-18.4454125678985,17.1136646200445,
-13.2954714863958));
#105264=CARTESIAN_POINT('Ctrl Pts',(-18.4930781369422,17.1075695618615,
-13.2982724892917));
#105265=CARTESIAN_POINT('Ctrl Pts',(-18.5207411502495,17.104585103667,-13.2998775388874));
#105266=CARTESIAN_POINT('Ctrl Pts',(-18.717162968989,17.0873032415419,-13.3111481511594));
#105267=CARTESIAN_POINT('Ctrl Pts',(-18.8870363146644,17.0927568789407,
-13.3201752962323));
#105268=CARTESIAN_POINT('Ctrl Pts',(-19.1572080616372,17.1341296375417,
-13.3351121649151));
#105269=CARTESIAN_POINT('Ctrl Pts',(-19.2586530023032,17.1574107146535,
-13.340876541378));
#105270=CARTESIAN_POINT('Ctrl Pts',(-19.3672203731698,17.190897326067,-13.3476076127931));
#105271=CARTESIAN_POINT('Ctrl Pts',(-19.3764579487496,17.1938161634937,
-13.3481849249218));
#105272=CARTESIAN_POINT('Ctrl Pts',(-19.3900688516309,17.1982198358758,
-13.349042793318));
#105273=CARTESIAN_POINT('Ctrl Pts',(-19.3944580260683,17.1996557922505,
-13.3493205510939));
#105274=CARTESIAN_POINT('Ctrl Pts',(-19.4022370979242,17.2022289912175,
-13.3498148714842));
#105275=CARTESIAN_POINT('Ctrl Pts',(-19.4056288496289,17.2033604723697,
-13.3500310925898));
#105276=CARTESIAN_POINT('Ctrl Pts',(-19.4128905138955,17.2058034097045,
-13.3504955196564));
#105277=CARTESIAN_POINT('Ctrl Pts',(-19.4167594425726,17.2071174589025,
-13.3507438722025));
#105278=CARTESIAN_POINT('Ctrl Pts',(-19.4273710736423,17.2107559095394,
-13.3514275059744));
#105279=CARTESIAN_POINT('Ctrl Pts',(-19.4341057994913,17.2131031724918,
-13.3518641066235));
#105280=CARTESIAN_POINT('Ctrl Pts',(-19.4695225453469,17.2256480819157,
-13.3541740312793));
#105281=CARTESIAN_POINT('Ctrl Pts',(-19.4979924247592,17.2364289059917,
-13.356079057898));
#105282=CARTESIAN_POINT('Ctrl Pts',(-19.6765791196524,17.3084954324587,
-13.3682924914236));
#105283=CARTESIAN_POINT('Ctrl Pts',(-19.8194667209514,17.3862424093955,
-13.3792084853915));
#105284=CARTESIAN_POINT('Ctrl Pts',(-20.0499071873122,17.5483562663366,
-13.3976307427178));
#105285=CARTESIAN_POINT('Ctrl Pts',(-20.1417396488845,17.6253539665135,
-13.4052583534821));
#105286=CARTESIAN_POINT('Ctrl Pts',(-20.2377288048237,17.7207867658016,
-13.4135235396185));
#105287=CARTESIAN_POINT('Ctrl Pts',(-20.2487462301813,17.7319869233607,
-13.4144773462716));
#105288=CARTESIAN_POINT('Ctrl Pts',(-20.2652268074862,17.7491181839616,
-13.4159122741625));
#105289=CARTESIAN_POINT('Ctrl Pts',(-20.2707822499671,17.7549593759034,
-13.4163974120406));
#105290=CARTESIAN_POINT('Ctrl Pts',(-20.2806777383223,17.7654835745531,
-13.4172642015325));
#105291=CARTESIAN_POINT('Ctrl Pts',(-20.2850301952312,17.7701547281809,
-13.4176463858278));
#105292=CARTESIAN_POINT('Ctrl Pts',(-20.2942209541851,17.7801083598774,
-13.4184554450099));
#105293=CARTESIAN_POINT('Ctrl Pts',(-20.2990537196481,17.7853958585207,
-13.4188820811029));
#105294=CARTESIAN_POINT('Ctrl Pts',(-20.3088371051771,17.7962095080493,
-13.4197482916651));
#105295=CARTESIAN_POINT('Ctrl Pts',(-20.3137857009629,17.8017373612013,
-13.4201877778931));
#105296=CARTESIAN_POINT('Ctrl Pts',(-20.3355743552209,17.826335477678,-13.4221289725536));
#105297=CARTESIAN_POINT('Ctrl Pts',(-20.3520993606331,17.8456828954844,
-13.4236175747887));
#105298=CARTESIAN_POINT('Ctrl Pts',(-20.4222714004769,17.9309041675784,
-13.4300186951382));
#105299=CARTESIAN_POINT('Ctrl Pts',(-20.4722775254316,17.999678774767,-13.4347859189593));
#105300=CARTESIAN_POINT('Ctrl Pts',(-20.5551898586189,18.1294624410505,
-13.4432735653916));
#105301=CARTESIAN_POINT('Ctrl Pts',(-20.5894925754731,18.1894307911714,
-13.4470186963147));
#105302=CARTESIAN_POINT('Ctrl Pts',(-20.6594231137151,18.3268692777156,
-13.4553933096343));
#105303=CARTESIAN_POINT('Ctrl Pts',(-20.6934048953441,18.4049868972709,
-13.4600145695703));
#105304=CARTESIAN_POINT('Ctrl Pts',(-20.722580578415,18.4848896205462,-13.4647888589437));
#105305=CARTESIAN_POINT('',(-20.8509991540684,19.2091074689689,-12.4890563034288));
#105306=CARTESIAN_POINT('Ctrl Pts',(-20.7225806137986,18.4848897174502,
-13.2445592988469));
#105307=CARTESIAN_POINT('Ctrl Pts',(-20.69626082822,18.4128083592617,-13.2399327222378));
#105308=CARTESIAN_POINT('Ctrl Pts',(-20.6660544393632,18.342259704581,-13.2353061456286));
#105309=CARTESIAN_POINT('Ctrl Pts',(-20.6321742240321,18.2736507506697,
-13.2306795690195));
#105310=CARTESIAN_POINT('Ctrl Pts',(-20.6214444484106,18.251922474332,-13.2292143443027));
#105311=CARTESIAN_POINT('Ctrl Pts',(-20.6103465313864,18.2303885369089,
-13.227749119586));
#105312=CARTESIAN_POINT('Ctrl Pts',(-20.598888138009,18.209061262994,-13.2262838948692));
#105313=CARTESIAN_POINT('Ctrl Pts',(-20.5645713376047,18.145188102246,-13.2218956859383));
#105314=CARTESIAN_POINT('Ctrl Pts',(-20.5269022333029,18.0829553476818,
-13.2175074770074));
#105315=CARTESIAN_POINT('Ctrl Pts',(-20.4860618340581,18.0227372640543,
-13.2131192680765));
#105316=CARTESIAN_POINT('Ctrl Pts',(-20.4452820487372,17.9626085540473,
-13.2087375719752));
#105317=CARTESIAN_POINT('Ctrl Pts',(-20.4013405804882,17.9044889751324,
-13.2043558758739));
#105318=CARTESIAN_POINT('Ctrl Pts',(-20.3544642120277,17.8487280970608,
-13.1999741797727));
#105319=CARTESIAN_POINT('Ctrl Pts',(-20.3076429270307,17.7930327424586,
-13.195597632513));
#105320=CARTESIAN_POINT('Ctrl Pts',(-20.2578939016345,17.7396909501819,
-13.1912210852534));
#105321=CARTESIAN_POINT('Ctrl Pts',(-20.2054860875596,17.6890217826399,
-13.1868445379937));
#105322=CARTESIAN_POINT('Ctrl Pts',(-20.1531115097587,17.6383847487476,
-13.1824707662768));
#105323=CARTESIAN_POINT('Ctrl Pts',(-20.0980818347927,17.5904173110763,
-13.1780969945598));
#105324=CARTESIAN_POINT('Ctrl Pts',(-20.040704044844,17.5454029481329,-13.1737232228428));
#105325=CARTESIAN_POINT('Ctrl Pts',(-19.9833437151495,17.5004022832114,
-13.1693507820792));
#105326=CARTESIAN_POINT('Ctrl Pts',(-19.9236370683463,17.4583532065245,
-13.1649783413157));
#105327=CARTESIAN_POINT('Ctrl Pts',(-19.8619241653155,17.419498931818,-13.1606059005521));
#105328=CARTESIAN_POINT('Ctrl Pts',(-19.800209684279,17.3806436636034,-13.1562333479848));
#105329=CARTESIAN_POINT('Ctrl Pts',(-19.7364892544384,17.3449836148752,
-13.1518607954174));
#105330=CARTESIAN_POINT('Ctrl Pts',(-19.6711304798848,17.3127177597441,
-13.1474882428501));
#105331=CARTESIAN_POINT('Ctrl Pts',(-19.6057038735297,17.2804184178915,
-13.1431111522827));
#105332=CARTESIAN_POINT('Ctrl Pts',(-19.5386359610928,17.251520516779,-13.1387340617154));
#105333=CARTESIAN_POINT('Ctrl Pts',(-19.4703166749593,17.2261758883526,
-13.1343569711481));
#105334=CARTESIAN_POINT('Ctrl Pts',(-19.401960077128,17.200817418284,-13.1299774900891));
#105335=CARTESIAN_POINT('Ctrl Pts',(-19.3323512055622,17.1790162288383,
-13.1255980090302));
#105336=CARTESIAN_POINT('Ctrl Pts',(-19.2618949953256,17.1608741809562,
-13.1212185279712));
#105337=CARTESIAN_POINT('Ctrl Pts',(-19.1913139019294,17.1426999764159,
-13.1168312843115));
#105338=CARTESIAN_POINT('Ctrl Pts',(-19.1198829437749,17.1281979613856,
-13.1124440406518));
#105339=CARTESIAN_POINT('Ctrl Pts',(-19.0480164983068,17.1174187049959,
-13.108056796992));
#105340=CARTESIAN_POINT('Ctrl Pts',(-18.9991542404234,17.1100898493376,
-13.1050738940573));
#105341=CARTESIAN_POINT('Ctrl Pts',(-18.950090817836,17.1044808253816,-13.1020909911225));
#105342=CARTESIAN_POINT('Ctrl Pts',(-18.9009566611239,17.1005937658104,
-13.0991080881877));
#105343=CARTESIAN_POINT('Ctrl Pts',(-18.8286744078925,17.0948754337364,
-13.0947198792568));
#105344=CARTESIAN_POINT('Ctrl Pts',(-18.7559569381435,17.0928637794812,
-13.0903316703259));
#105345=CARTESIAN_POINT('Ctrl Pts',(-18.6832169260195,17.0946091855716,
-13.085943461395));
#105346=CARTESIAN_POINT('Ctrl Pts',(-18.6105848721339,17.0963520011899,
-13.0815617652938));
#105347=CARTESIAN_POINT('Ctrl Pts',(-18.537930820542,17.1018407963575,-13.0771800691925));
#105348=CARTESIAN_POINT('Ctrl Pts',(-18.4656714572671,17.1110740981752,
-13.0727983730912));
#105349=CARTESIAN_POINT('Ctrl Pts',(-18.3934970044947,17.1202965501284,
-13.0684218258316));
#105350=CARTESIAN_POINT('Ctrl Pts',(-18.3217167948296,17.1332547070803,
-13.064045278572));
#105351=CARTESIAN_POINT('Ctrl Pts',(-18.2507446877305,17.1498951256272,
-13.0596687313123));
#105352=CARTESIAN_POINT('Ctrl Pts',(-18.1798175901102,17.1665249910625,
-13.0552949595953));
#105353=CARTESIAN_POINT('Ctrl Pts',(-18.1096980467015,17.1868323748369,
-13.0509211878784));
#105354=CARTESIAN_POINT('Ctrl Pts',(-18.0407905817002,17.2107125950553,
-13.0465474161614));
#105355=CARTESIAN_POINT('Ctrl Pts',(-17.9719040854719,17.2345855484424,
-13.0421749753978));
#105356=CARTESIAN_POINT('Ctrl Pts',(-17.9042293909005,17.2620290219354,
-13.0378025346343));
#105357=CARTESIAN_POINT('Ctrl Pts',(-17.8381550707619,17.2928887251365,
-13.0334300938707));
#105358=CARTESIAN_POINT('Ctrl Pts',(-17.7720790610957,17.3237492174237,
-13.0290575413034));
#105359=CARTESIAN_POINT('Ctrl Pts',(-17.7076039433213,17.3580259069127,
-13.0246849887361));
#105360=CARTESIAN_POINT('Ctrl Pts',(-17.6450960002997,17.3955173976497,
-13.0203124361687));
#105361=CARTESIAN_POINT('Ctrl Pts',(-17.5825231841771,17.4330477984699,
-13.0159353456014));
#105362=CARTESIAN_POINT('Ctrl Pts',(-17.5219220335749,17.4737994133219,
-13.0115582550341));
#105363=CARTESIAN_POINT('Ctrl Pts',(-17.4636312781365,17.5175265545304,
-13.0071811644667));
#105364=CARTESIAN_POINT('Ctrl Pts',(-17.405308687953,17.5612775767536,-13.0028016834078));
#105365=CARTESIAN_POINT('Ctrl Pts',(-17.3492993758003,17.6080070515429,
-12.9984222023489));
#105366=CARTESIAN_POINT('Ctrl Pts',(-17.2959081742794,17.6574296279873,
-12.9940427212899));
#105367=CARTESIAN_POINT('Ctrl Pts',(-17.2424223372123,17.7069398056167,
-12.9896554776302));
#105368=CARTESIAN_POINT('Ctrl Pts',(-17.1915642147117,17.7591522715469,
-12.9852682339705));
#105369=CARTESIAN_POINT('Ctrl Pts',(-17.1436006220652,17.8137459720349,
-12.9808809903108));
#105370=CARTESIAN_POINT('Ctrl Pts',(-17.1109900008265,17.8508644277303,
-12.9778980873759));
#105371=CARTESIAN_POINT('Ctrl Pts',(-17.0797165992412,17.8890829433879,
-12.9749151844411));
#105372=CARTESIAN_POINT('Ctrl Pts',(-17.0498528101567,17.9282930019124,
-12.9719322815063));
#105373=CARTESIAN_POINT('Ctrl Pts',(-17.0059195850954,17.9859757132705,
-12.9675440725754));
#105374=CARTESIAN_POINT('Ctrl Pts',(-16.9648675150387,18.046030727246,-12.9631558636445));
#105375=CARTESIAN_POINT('Ctrl Pts',(-16.9269623364049,18.1081383212983,
-12.9587676547136));
#105376=CARTESIAN_POINT('Ctrl Pts',(-16.889113415341,18.1701537373834,-12.9543859586123));
#105377=CARTESIAN_POINT('Ctrl Pts',(-16.8544023633226,18.2342152777403,
-12.9500042625111));
#105378=CARTESIAN_POINT('Ctrl Pts',(-16.8230534861161,18.2999717781127,
-12.9456225664098));
#105379=CARTESIAN_POINT('Ctrl Pts',(-16.7917414463352,18.3656510093642,
-12.9412460191502));
#105380=CARTESIAN_POINT('Ctrl Pts',(-16.7637839395866,18.4330208108152,
-12.9368694718905));
#105381=CARTESIAN_POINT('Ctrl Pts',(-16.7393600427009,18.5017042642551,
-12.9324929246309));
#105382=CARTESIAN_POINT('Ctrl Pts',(-16.7149516350957,18.5703441596469,
-12.9281191529139));
#105383=CARTESIAN_POINT('Ctrl Pts',(-16.694072552212,18.6402956006724,-12.9237453811969));
#105384=CARTESIAN_POINT('Ctrl Pts',(-16.6768537344171,18.7111617841757,
-12.91937160948));
#105385=CARTESIAN_POINT('Ctrl Pts',(-16.6596401563663,18.7820064028615,
-12.9149991687164));
#105386=CARTESIAN_POINT('Ctrl Pts',(-16.6460847459306,18.8537647429385,
-12.9106267279528));
#105387=CARTESIAN_POINT('Ctrl Pts',(-16.6362680963764,18.9260265617294,
-12.9062542871893));
#105388=CARTESIAN_POINT('Ctrl Pts',(-16.6264511958094,18.998290228263,-12.9018817346219));
#105389=CARTESIAN_POINT('Ctrl Pts',(-16.620373308882,19.0710569208143,-12.8975091820546));
#105390=CARTESIAN_POINT('Ctrl Pts',(-16.6180633554341,19.1439096416525,
-12.8931366294872));
#105391=CARTESIAN_POINT('Ctrl Pts',(-16.6157510046294,19.2168379717925,
-12.8887595389199));
#105392=CARTESIAN_POINT('Ctrl Pts',(-16.6172144102078,19.2898520253128,
-12.8843824483526));
#105393=CARTESIAN_POINT('Ctrl Pts',(-16.6224303356468,19.3625339981098,
-12.8800053577853));
#105394=CARTESIAN_POINT('Ctrl Pts',(-16.6276491096962,19.4352556652298,
-12.8756258767263));
#105395=CARTESIAN_POINT('Ctrl Pts',(-16.6366244245267,19.5076444114932,
-12.8712463956674));
#105396=CARTESIAN_POINT('Ctrl Pts',(-16.6492813452851,19.5792894658875,
-12.8668669146084));
#105397=CARTESIAN_POINT('Ctrl Pts',(-16.6619607003506,19.6510615106598,
-12.8624796709487));
#105398=CARTESIAN_POINT('Ctrl Pts',(-16.678334584287,19.7220867607307,-12.858092427289));
#105399=CARTESIAN_POINT('Ctrl Pts',(-16.698277463759,19.791967086366,-12.8537051836293));
#105400=CARTESIAN_POINT('Ctrl Pts',(-16.7118367001087,19.8394789741459,
-12.8507222806944));
#105401=CARTESIAN_POINT('Ctrl Pts',(-16.7270447244344,19.88646191341,-12.8477393777596));
#105402=CARTESIAN_POINT('Ctrl Pts',(-16.7438494759074,19.9327962949848,
-12.8447564748248));
#105403=CARTESIAN_POINT('Ctrl Pts',(-16.7685712862064,20.0009597422968,
-12.8403682658939));
#105404=CARTESIAN_POINT('Ctrl Pts',(-16.7968473421402,20.0679846766149,
-12.835980056963));
#105405=CARTESIAN_POINT('Ctrl Pts',(-16.8285526457323,20.1334745959182,
-12.8315918480321));
#105406=CARTESIAN_POINT('Ctrl Pts',(-16.8602108933972,20.1988673173228,
-12.8272101519309));
#105407=CARTESIAN_POINT('Ctrl Pts',(-16.8952880767684,20.2627291156991,
-12.8228284558296));
#105408=CARTESIAN_POINT('Ctrl Pts',(-16.9336103347365,20.3246813068434,
-12.8184467597283));
#105409=CARTESIAN_POINT('Ctrl Pts',(-16.9718875610016,20.3865606992326,
-12.8140702124687));
#105410=CARTESIAN_POINT('Ctrl Pts',(-17.0134020343728,20.4465345337929,
-12.8096936652091));
#105411=CARTESIAN_POINT('Ctrl Pts',(-17.0579337571751,20.5042482165705,
-12.8053171179494));
#105412=CARTESIAN_POINT('Ctrl Pts',(-17.102437238606,20.5619252981693,-12.8009433462325));
#105413=CARTESIAN_POINT('Ctrl Pts',(-17.1499538788911,20.617344690981,-12.7965695745155));
#105414=CARTESIAN_POINT('Ctrl Pts',(-17.200220904909,20.6701815128564,-12.7921958027985));
#105415=CARTESIAN_POINT('Ctrl Pts',(-17.2504726345021,20.7230022563095,
-12.787823362035));
#105416=CARTESIAN_POINT('Ctrl Pts',(-17.3034727559332,20.7732416397748,
-12.7834509212714));
#105417=CARTESIAN_POINT('Ctrl Pts',(-17.3589199436394,20.8206098404891,
-12.7790784805079));
#105418=CARTESIAN_POINT('Ctrl Pts',(-17.4143685491363,20.8679792524135,
-12.7747059279405));
#105419=CARTESIAN_POINT('Ctrl Pts',(-17.4722639770756,20.9124770240216,
-12.7703333753732));
#105420=CARTESIAN_POINT('Ctrl Pts',(-17.5322712521179,20.9538531253418,
-12.7659608228058));
#105421=CARTESIAN_POINT('Ctrl Pts',(-17.5923408049737,20.9952721683407,
-12.7615837322385));
#105422=CARTESIAN_POINT('Ctrl Pts',(-17.6545261829437,21.0335627981877,
-12.7572066416712));
#105423=CARTESIAN_POINT('Ctrl Pts',(-17.7184635014066,21.068518403684,-12.7528295511039));
#105424=CARTESIAN_POINT('Ctrl Pts',(-17.7824357384122,21.1034930997338,
-12.7484500700449));
#105425=CARTESIAN_POINT('Ctrl Pts',(-17.8481613859397,21.135128935727,-12.744070588986));
#105426=CARTESIAN_POINT('Ctrl Pts',(-17.9152544897586,21.163266577458,-12.7396911079271));
#105427=CARTESIAN_POINT('Ctrl Pts',(-17.9824665156537,21.1914540929701,
-12.7353038642673));
#105428=CARTESIAN_POINT('Ctrl Pts',(-18.0510503837933,21.2161308685658,
-12.7309166206076));
#105429=CARTESIAN_POINT('Ctrl Pts',(-18.1206033812628,21.2371869578402,
-12.7265293769479));
#105430=CARTESIAN_POINT('Ctrl Pts',(-18.1678927174314,21.2515030695869,
-12.7235464740131));
#105431=CARTESIAN_POINT('Ctrl Pts',(-18.2156297492658,21.2641465017728,
-12.7205635710783));
#105432=CARTESIAN_POINT('Ctrl Pts',(-18.2636857248404,21.275096287139,-12.7175806681434));
#105433=CARTESIAN_POINT('Ctrl Pts',(-18.334381843959,21.2912047381968,-12.7131924592126));
#105434=CARTESIAN_POINT('Ctrl Pts',(-18.4060444995739,21.3037083756574,
-12.7088042502817));
#105435=CARTESIAN_POINT('Ctrl Pts',(-18.4782726371993,21.3124976840137,
-12.7044160413508));
#105436=CARTESIAN_POINT('Ctrl Pts',(-18.5503935762929,21.3212739475792,
-12.7000343452495));
#105437=CARTESIAN_POINT('Ctrl Pts',(-18.6230778564461,21.3263467676749,
-12.6956526491482));
#105438=CARTESIAN_POINT('Ctrl Pts',(-18.6959129564506,21.3276573594027,
-12.691270953047));
#105439=CARTESIAN_POINT('Ctrl Pts',(-18.7686624694161,21.3289664110809,
-12.6868944057873));
#105440=CARTESIAN_POINT('Ctrl Pts',(-18.8415619702678,21.3265220079374,
-12.6825178585277));
#105441=CARTESIAN_POINT('Ctrl Pts',(-18.9141942210374,21.3203171982195,
-12.6781413112681));
#105442=CARTESIAN_POINT('Ctrl Pts',(-18.9867804094892,21.3141163235018,
-12.6737675395511));
#105443=CARTESIAN_POINT('Ctrl Pts',(-19.0590992046968,21.3041598149105,
-12.6693937678341));
#105444=CARTESIAN_POINT('Ctrl Pts',(-19.1307351980796,21.2904927705103,
-12.6650199961171));
#105445=CARTESIAN_POINT('Ctrl Pts',(-19.2023493923891,21.2768298850377,
-12.6606475553536));
#105446=CARTESIAN_POINT('Ctrl Pts',(-19.2732807238325,21.2594587957697,
-12.65627511459));
#105447=CARTESIAN_POINT('Ctrl Pts',(-19.3431223955192,21.2384759942542,
-12.6519026738265));
#105448=CARTESIAN_POINT('Ctrl Pts',(-19.4129658530652,21.2174926562061,
-12.6475301212592));
#105449=CARTESIAN_POINT('Ctrl Pts',(-19.4817191341324,21.1928975632637,
-12.6431575686918));
#105450=CARTESIAN_POINT('Ctrl Pts',(-19.5489906872852,21.1648370401951,
-12.6387850161245));
#105451=CARTESIAN_POINT('Ctrl Pts',(-19.6163320573932,21.1367473948573,
-12.6344079255571));
#105452=CARTESIAN_POINT('Ctrl Pts',(-19.6821881831272,21.1051853247309,
-12.6300308349898));
#105453=CARTESIAN_POINT('Ctrl Pts',(-19.7461883733219,21.0703449644732,
-12.6256537444225));
#105454=CARTESIAN_POINT('Ctrl Pts',(-19.8102235163959,21.0354855766017,
-12.6212742633636));
#105455=CARTESIAN_POINT('Ctrl Pts',(-19.8724002944077,20.9973445863424,
-12.6168947823046));
#105456=CARTESIAN_POINT('Ctrl Pts',(-19.932375822801,20.9561602755409,-12.6125153012457));
#105457=CARTESIAN_POINT('Ctrl Pts',(-19.9924576574157,20.9149029658251,
-12.608128057586));
#105458=CARTESIAN_POINT('Ctrl Pts',(-20.0503300675354,20.87059185695,-12.6037408139262));
#105459=CARTESIAN_POINT('Ctrl Pts',(-20.1056826247701,20.8235060548425,
-12.5993535702665));
#105460=CARTESIAN_POINT('Ctrl Pts',(-20.1433170299302,20.7914922465863,
-12.5963706673317));
#105461=CARTESIAN_POINT('Ctrl Pts',(-20.1797873054598,20.758196607403,-12.5933877643969));
#105462=CARTESIAN_POINT('Ctrl Pts',(-20.2150061302367,20.7237160481073,
-12.590404861462));
#105463=CARTESIAN_POINT('Ctrl Pts',(-20.2660558507878,20.6737364440846,
-12.5860811407752));
#105464=CARTESIAN_POINT('Ctrl Pts',(-20.3146860821103,20.6210584681426,
-12.5817574200883));
#105465=CARTESIAN_POINT('Ctrl Pts',(-20.3605919747978,20.5659492785797,
-12.5774336994015));
#105466=CARTESIAN_POINT('Ctrl Pts',(-20.4064369112151,20.5109132659108,
-12.5731157199794));
#105467=CARTESIAN_POINT('Ctrl Pts',(-20.4495643625503,20.453452815078,-12.5687977405574));
#105468=CARTESIAN_POINT('Ctrl Pts',(-20.4897052944035,20.3938727400712,
-12.5644797611354));
#105469=CARTESIAN_POINT('Ctrl Pts',(-20.5298070691323,20.3343507849011,
-12.5601659938641));
#105470=CARTESIAN_POINT('Ctrl Pts',(-20.5669278234435,20.2727137148021,
-12.5558522265928));
#105471=CARTESIAN_POINT('Ctrl Pts',(-20.600839132399,20.2092988799672,-12.5515384593216));
#105472=CARTESIAN_POINT('Ctrl Pts',(-20.6347293023106,20.1459235755726,
-12.5472273810918));
#105473=CARTESIAN_POINT('Ctrl Pts',(-20.6654137615196,20.0807731423998,
-12.542916302862));
#105474=CARTESIAN_POINT('Ctrl Pts',(-20.6927087374024,20.0142117292615,
-12.5386052246321));
#105475=CARTESIAN_POINT('Ctrl Pts',(-20.720007692024,19.9476406135877,-12.5342935179843));
#105476=CARTESIAN_POINT('Ctrl Pts',(-20.7439159714602,19.8796585609649,
-12.5299818113365));
#105477=CARTESIAN_POINT('Ctrl Pts',(-20.7642975065946,19.8106507606231,
-12.5256701046887));
#105478=CARTESIAN_POINT('Ctrl Pts',(-20.7846795217662,19.7416413349712,
-12.5213582964892));
#105479=CARTESIAN_POINT('Ctrl Pts',(-20.8015344966335,19.671606594183,-12.5170464882896));
#105480=CARTESIAN_POINT('Ctrl Pts',(-20.8147766394152,19.6009456075709,
-12.5127346800901));
#105481=CARTESIAN_POINT('Ctrl Pts',(-20.8280335437791,19.5302058521392,
-12.5084180653338));
#105482=CARTESIAN_POINT('Ctrl Pts',(-20.8376694934189,19.4588389489561,
-12.5041014505775));
#105483=CARTESIAN_POINT('Ctrl Pts',(-20.8436502754156,19.3872518522996,
-12.4997848358213));
#105484=CARTESIAN_POINT('Ctrl Pts',(-20.8486051622892,19.3279442290249,
-12.4962086583571));
#105485=CARTESIAN_POINT('Ctrl Pts',(-20.8510522363726,19.2684857254966,
-12.4926324808929));
#105486=CARTESIAN_POINT('Ctrl Pts',(-20.8509991540684,19.2091074689689,
-12.4890563034288));
#105487=CARTESIAN_POINT('Ctrl Pts',(-20.8516474773841,19.2091064840258,
-12.4890562790225));
#105488=CARTESIAN_POINT('Ctrl Pts',(-20.8529701850388,19.0661177649361,
-12.4804472042752));
#105489=CARTESIAN_POINT('Ctrl Pts',(-20.8300642588143,18.8192068783604,
-12.4655558065448));
#105490=CARTESIAN_POINT('Ctrl Pts',(-20.7608947058963,18.581811275593,-12.4506644088145));
#105491=CARTESIAN_POINT('Ctrl Pts',(-20.7242505411024,18.4842642021379,
-12.4443820858314));
#105492=CARTESIAN_POINT('Origin',(-18.734,19.211,0.));
#105493=CARTESIAN_POINT('',(-20.7225806143616,18.4848897189921,-11.6425493859455));
#105494=CARTESIAN_POINT('',(-20.7225806137507,18.4848897173191,-11.8674650369494));
#105495=CARTESIAN_POINT('',(-20.7225806137986,18.4848897174502,0.));
#105496=CARTESIAN_POINT('',(-20.8509993992231,19.2125948947384,-11.912063495998));
#105497=CARTESIAN_POINT('Ctrl Pts',(-20.7225806137507,18.4848897173191,
-11.8674650369494));
#105498=CARTESIAN_POINT('Ctrl Pts',(-20.7358715688534,18.5212893335838,
-11.869979723211));
#105499=CARTESIAN_POINT('Ctrl Pts',(-20.7481612761736,18.5580488153306,
-11.8724726491891));
#105500=CARTESIAN_POINT('Ctrl Pts',(-20.7623061769257,18.6045674671939,
-11.8755657388135));
#105501=CARTESIAN_POINT('Ctrl Pts',(-20.765110754078,18.6140280798097,-11.8761916412424));
#105502=CARTESIAN_POINT('Ctrl Pts',(-20.7833787104828,18.6772702539463,
-11.8803545618301));
#105503=CARTESIAN_POINT('Ctrl Pts',(-20.7967715338951,18.7316305576149,
-11.8838304061372));
#105504=CARTESIAN_POINT('Ctrl Pts',(-20.8104072908029,18.7982453194696,
-11.8879694996));
#105505=CARTESIAN_POINT('Ctrl Pts',(-20.8127188548269,18.8100491357361,
-11.8886984336853));
#105506=CARTESIAN_POINT('Ctrl Pts',(-20.8163752084312,18.8296021335995,
-11.8898986409805));
#105507=CARTESIAN_POINT('Ctrl Pts',(-20.8177776152043,18.8373401357374,
-11.8903717414125));
#105508=CARTESIAN_POINT('Ctrl Pts',(-20.8202374454822,18.8513573114023,
-11.8912254139216));
#105509=CARTESIAN_POINT('Ctrl Pts',(-20.821309713366,18.8576337533753,-11.8916064539954));
#105510=CARTESIAN_POINT('Ctrl Pts',(-20.823336457162,18.8698283388792,-11.8923444756629));
#105511=CARTESIAN_POINT('Ctrl Pts',(-20.8242941443647,18.8757458803418,
-11.8927015558131));
#105512=CARTESIAN_POINT('Ctrl Pts',(-20.826339673241,18.8887347715827,-11.8934830704994));
#105513=CARTESIAN_POINT('Ctrl Pts',(-20.8274168317906,18.895807747638,-11.8939071640037));
#105514=CARTESIAN_POINT('Ctrl Pts',(-20.8299772014903,18.913212309321,-11.8949471940112));
#105515=CARTESIAN_POINT('Ctrl Pts',(-20.8314199118356,18.9235497310235,
-11.8955618545989));
#105516=CARTESIAN_POINT('Ctrl Pts',(-20.8449846042971,19.0262893038818,
-11.9016414009509));
#105517=CARTESIAN_POINT('Ctrl Pts',(-20.8510696179088,19.1193894235361,
-11.9069087635312));
#105518=CARTESIAN_POINT('Ctrl Pts',(-20.8509993992231,19.2125948947384,
-11.912063495998));
#105519=CARTESIAN_POINT('Ctrl Pts',(-20.8509994011049,19.2125923949245,
-11.9120633577456));
#105520=CARTESIAN_POINT('Ctrl Pts',(-20.8508903570202,19.3575603663925,
-11.9200808205576));
#105521=CARTESIAN_POINT('Ctrl Pts',(-20.8358914523054,19.5021322706615,
-11.9277753972783));
#105522=CARTESIAN_POINT('Ctrl Pts',(-20.7926402019966,19.709104411674,-11.9395053011385));
#105523=CARTESIAN_POINT('Ctrl Pts',(-20.7759875264153,19.7734879564716,
-11.9432643032825));
#105524=CARTESIAN_POINT('Ctrl Pts',(-20.7524080810177,19.8496660435697,
-11.947959439339));
#105525=CARTESIAN_POINT('Ctrl Pts',(-20.7483605177477,19.8623195691038,
-11.9487477000343));
#105526=CARTESIAN_POINT('Ctrl Pts',(-20.7425481574265,19.8799176689914,
-11.9498567939057));
#105527=CARTESIAN_POINT('Ctrl Pts',(-20.7408835583365,19.8848953409272,
-11.9501719417593));
#105528=CARTESIAN_POINT('Ctrl Pts',(-20.7380219445164,19.8933478240683,
-11.9507096166996));
#105529=CARTESIAN_POINT('Ctrl Pts',(-20.7368343462604,19.8968258440078,
-11.9509315890967));
#105530=CARTESIAN_POINT('Ctrl Pts',(-20.7345445651943,19.9034750637692,
-11.9513573813501));
#105531=CARTESIAN_POINT('Ctrl Pts',(-20.7334438881852,19.9066467558357,
-11.9515611071857));
#105532=CARTESIAN_POINT('Ctrl Pts',(-20.7305162330582,19.9150186870069,
-11.9521004766321));
#105533=CARTESIAN_POINT('Ctrl Pts',(-20.7286764966813,19.9202143910975,
-11.9524368680168));
#105534=CARTESIAN_POINT('Ctrl Pts',(-20.722118593999,19.9385075683665,-11.9536269312589));
#105535=CARTESIAN_POINT('Ctrl Pts',(-20.7172916623693,19.9515653005,-11.9544867064343));
#105536=CARTESIAN_POINT('Ctrl Pts',(-20.6531107493891,20.1200576144672,
-11.9657061258321));
#105537=CARTESIAN_POINT('Ctrl Pts',(-20.5757664590092,20.2680063725952,
-11.9768935660573));
#105538=CARTESIAN_POINT('Ctrl Pts',(-20.4366046845345,20.4716641432207,
-11.9930979794031));
#105539=CARTESIAN_POINT('Ctrl Pts',(-20.387563583073,20.5353361806168,-11.9983096747123));
#105540=CARTESIAN_POINT('Ctrl Pts',(-20.3092874391038,20.6258163447576,
-12.0058901418974));
#105541=CARTESIAN_POINT('Ctrl Pts',(-20.2827306186546,20.6548384915281,
-12.0083517684621));
#105542=CARTESIAN_POINT('Ctrl Pts',(-20.2369236281096,20.7021787174121,
-12.0124188879455));
#105543=CARTESIAN_POINT('Ctrl Pts',(-20.2181103922107,20.7209039186198,
-12.014042124923));
#105544=CARTESIAN_POINT('Ctrl Pts',(-20.1918823967089,20.7460451938731,
-12.0162427451026));
#105545=CARTESIAN_POINT('Ctrl Pts',(-20.184768487642,20.7527702909866,-12.0168335464193));
#105546=CARTESIAN_POINT('Ctrl Pts',(-20.1732500031756,20.7635089144527,
-12.0177805123631));
#105547=CARTESIAN_POINT('Ctrl Pts',(-20.1688747467957,20.7675535529602,
-12.0181380111008));
#105548=CARTESIAN_POINT('Ctrl Pts',(-20.1597234101342,20.7759419911736,
-12.0188812168942));
#105549=CARTESIAN_POINT('Ctrl Pts',(-20.1549444128617,20.7802825287135,
-12.019266783022));
#105550=CARTESIAN_POINT('Ctrl Pts',(-20.1438651762256,20.7902531695571,
-12.0201548315509));
#105551=CARTESIAN_POINT('Ctrl Pts',(-20.1375509102739,20.7958675762083,
-12.0206566496767));
#105552=CARTESIAN_POINT('Ctrl Pts',(-20.1204817448211,20.8108628165386,
-12.0220018378533));
#105553=CARTESIAN_POINT('Ctrl Pts',(-20.1096652052803,20.8201730541798,
-12.0228422763222));
#105554=CARTESIAN_POINT('Ctrl Pts',(-20.0094125557049,20.9047149290194,
-12.0305251328716));
#105555=CARTESIAN_POINT('Ctrl Pts',(-19.913979394313,20.9725338046926,-12.0370506413779));
#105556=CARTESIAN_POINT('Ctrl Pts',(-19.6733916488256,21.1151350699243,
-12.0523612625821));
#105557=CARTESIAN_POINT('Ctrl Pts',(-19.5242711950226,21.1816969838733,
-12.060963258126));
#105558=CARTESIAN_POINT('Ctrl Pts',(-19.3380509824021,21.2402523996148,
-12.0721724245961));
#105559=CARTESIAN_POINT('Ctrl Pts',(-19.3068642141171,21.2492760418074,
-12.0740659240699));
#105560=CARTESIAN_POINT('Ctrl Pts',(-19.2684884657816,21.2594295076322,
-12.0764294908508));
#105561=CARTESIAN_POINT('Ctrl Pts',(-19.2614832987398,21.2612445546577,
-12.0768622971979));
#105562=CARTESIAN_POINT('Ctrl Pts',(-19.2504861690386,21.2640338334509,
-12.0775440650814));
#105563=CARTESIAN_POINT('Ctrl Pts',(-19.2465003652833,21.2650324386501,
-12.0777916423319));
#105564=CARTESIAN_POINT('Ctrl Pts',(-19.239044257761,21.26687744216,-12.0782557108702));
#105565=CARTESIAN_POINT('Ctrl Pts',(-19.2355747105171,21.2677266635586,
-12.0784720370395));
#105566=CARTESIAN_POINT('Ctrl Pts',(-19.2276491610404,21.2696453082994,
-12.0789670559725));
#105567=CARTESIAN_POINT('Ctrl Pts',(-19.2231918407841,21.2707090429421,
-12.0792460709584));
#105568=CARTESIAN_POINT('Ctrl Pts',(-19.2094782326545,21.2739347550957,
-12.0801063217819));
#105569=CARTESIAN_POINT('Ctrl Pts',(-19.2002109578109,21.2760488344306,
-12.08069020016));
#105570=CARTESIAN_POINT('Ctrl Pts',(-19.1166836618199,21.2945124389833,
-12.0859737007823));
#105571=CARTESIAN_POINT('Ctrl Pts',(-19.0416148126414,21.3069106466933,
-12.0908690648959));
#105572=CARTESIAN_POINT('Ctrl Pts',(-18.8155829400092,21.3318369175994,
-12.1057426640404));
#105573=CARTESIAN_POINT('Ctrl Pts',(-18.6637507285478,21.3322442579105,
-12.1158740241582));
#105574=CARTESIAN_POINT('Ctrl Pts',(-18.4580865450591,21.3106734585856,
-12.1291691800293));
#105575=CARTESIAN_POINT('Ctrl Pts',(-18.4032449808158,21.3027358384152,
-12.1326772615108));
#105576=CARTESIAN_POINT('Ctrl Pts',(-18.3149154988974,21.2863898039453,
-12.1382614599131));
#105577=CARTESIAN_POINT('Ctrl Pts',(-18.2812134722424,21.2792986332837,
-12.1403764763748));
#105578=CARTESIAN_POINT('Ctrl Pts',(-18.2371638692775,21.2689018452238,
-12.1431218803234));
#105579=CARTESIAN_POINT('Ctrl Pts',(-18.2266490042642,21.2663347949438,
-12.1437757988958));
#105580=CARTESIAN_POINT('Ctrl Pts',(-18.2094624986717,21.2619990340104,
-12.1448424078432));
#105581=CARTESIAN_POINT('Ctrl Pts',(-18.2027790982131,21.2602781614682,
-12.1452566338115));
#105582=CARTESIAN_POINT('Ctrl Pts',(-18.1898606024616,21.256884402527,-12.146056274025));
#105583=CARTESIAN_POINT('Ctrl Pts',(-18.1836245171632,21.2552156201765,
-12.1464418159959));
#105584=CARTESIAN_POINT('Ctrl Pts',(-18.1692466990184,21.2512975405058,
-12.1473296872615));
#105585=CARTESIAN_POINT('Ctrl Pts',(-18.1611105649305,21.2490279789796,
-12.1478313531342));
#105586=CARTESIAN_POINT('Ctrl Pts',(-18.1392737832821,21.2427955438061,
-12.149175863685));
#105587=CARTESIAN_POINT('Ctrl Pts',(-18.1255990886412,21.2387427722877,
-12.1500157814584));
#105588=CARTESIAN_POINT('Ctrl Pts',(-18.0002992283032,21.2002259690837,
-12.1576955283891));
#105589=CARTESIAN_POINT('Ctrl Pts',(-17.891658331607,21.1567138937895,-12.1642187007505));
#105590=CARTESIAN_POINT('Ctrl Pts',(-17.6417216234923,21.0317293321491,
-12.1795170892452));
#105591=CARTESIAN_POINT('Ctrl Pts',(-17.50517311852,20.9425022547793,-12.1881097439642));
#105592=CARTESIAN_POINT('Ctrl Pts',(-17.3550700894167,20.8176453786321,
-12.1993181973251));
#105593=CARTESIAN_POINT('Ctrl Pts',(-17.3304336058437,20.7961681876,-12.2012240685647));
#105594=CARTESIAN_POINT('Ctrl Pts',(-17.3009514224285,20.7692404683417,
-12.2036013977632));
#105595=CARTESIAN_POINT('Ctrl Pts',(-17.2956224480114,20.7643227601928,
-12.2040350811563));
#105596=CARTESIAN_POINT('Ctrl Pts',(-17.2873111949527,20.7565734897704,
-12.2047179265899));
#105597=CARTESIAN_POINT('Ctrl Pts',(-17.2843116651068,20.7537603968029,
-12.2049656971147));
#105598=CARTESIAN_POINT('Ctrl Pts',(-17.2787223597263,20.7484878034898,
-12.2054299294243));
#105599=CARTESIAN_POINT('Ctrl Pts',(-17.2761306053488,20.7460304829698,
-12.2056462248791));
#105600=CARTESIAN_POINT('Ctrl Pts',(-17.2702311954537,20.7404086574444,
-12.2061409118672));
#105601=CARTESIAN_POINT('Ctrl Pts',(-17.2669275897185,20.7372399866044,
-12.2064196239426));
#105602=CARTESIAN_POINT('Ctrl Pts',(-17.2568136745195,20.7274759935125,
-12.207278034215));
#105603=CARTESIAN_POINT('Ctrl Pts',(-17.2500374794555,20.7208457235827,
-12.2078603589001));
#105604=CARTESIAN_POINT('Ctrl Pts',(-17.1573428745015,20.6289204953568,
-12.2159230830404));
#105605=CARTESIAN_POINT('Ctrl Pts',(-17.0788605425881,20.5364632518845,
-12.2238920357722));
#105606=CARTESIAN_POINT('Ctrl Pts',(-16.9050472727718,20.292028949297,-12.2437081062179));
#105607=CARTESIAN_POINT('Ctrl Pts',(-16.8202527669139,20.1336528795698,
-12.2554516534286));
#105608=CARTESIAN_POINT('Ctrl Pts',(-16.7487232006562,19.9464089652028,
-12.2677649610291));
#105609=CARTESIAN_POINT('Ctrl Pts',(-16.7413640368456,19.9262288359775,
-12.2690742199382));
#105610=CARTESIAN_POINT('Ctrl Pts',(-16.7313506267608,19.8974152737031,
-12.2709190638132));
#105611=CARTESIAN_POINT('Ctrl Pts',(-16.7284427171872,19.8888719860025,
-12.271463033325));
#105612=CARTESIAN_POINT('Ctrl Pts',(-16.7235252790679,19.8741161470664,
-12.2723974326037));
#105613=CARTESIAN_POINT('Ctrl Pts',(-16.7214897159683,19.867912464607,-12.2727887183452));
#105614=CARTESIAN_POINT('Ctrl Pts',(-16.7176504287978,19.8560263161585,
-12.2735354783316));
#105615=CARTESIAN_POINT('Ctrl Pts',(-16.7158419482694,19.850345463094,-12.2738911061059));
#105616=CARTESIAN_POINT('Ctrl Pts',(-16.7112085858819,19.8355754444516,
-12.2748124537305));
#105617=CARTESIAN_POINT('Ctrl Pts',(-16.7084209400011,19.8264746680678,
-12.2753769482363));
#105618=CARTESIAN_POINT('Ctrl Pts',(-16.6991587323188,19.7954918679359,
-12.2772880897035));
#105619=CARTESIAN_POINT('Ctrl Pts',(-16.6929764876236,19.7735236082731,
-12.2786252095429));
#105620=CARTESIAN_POINT('Ctrl Pts',(-16.6417820048902,19.5796376772178,
-12.2902797451863));
#105621=CARTESIAN_POINT('Ctrl Pts',(-16.6182276133207,19.402790694168,-12.2998237830137));
#105622=CARTESIAN_POINT('Ctrl Pts',(-16.6164789542422,19.1396149196788,
-12.314149024606));
#105623=CARTESIAN_POINT('Ctrl Pts',(-16.6210856254121,19.054214320218,-12.3188318710045));
#105624=CARTESIAN_POINT('Ctrl Pts',(-16.6351115504586,18.9321503895753,
-12.325849763404));
#105625=CARTESIAN_POINT('Ctrl Pts',(-16.6403691389444,18.8950897931115,
-12.3280244807594));
#105626=CARTESIAN_POINT('Ctrl Pts',(-16.6478638698815,18.8507472641974,
-12.3307002934696));
#105627=CARTESIAN_POINT('Ctrl Pts',(-16.6491617299718,18.843310768482,-12.3311515531232));
#105628=CARTESIAN_POINT('Ctrl Pts',(-16.6512395090436,18.831770270929,-12.3318559762129));
#105629=CARTESIAN_POINT('Ctrl Pts',(-16.6519918644425,18.8276612817882,
-12.3321075998139));
#105630=CARTESIAN_POINT('Ctrl Pts',(-16.653408677252,18.820050577058,-12.3325752135234));
#105631=CARTESIAN_POINT('Ctrl Pts',(-16.654069818119,18.8165483026953,-12.3327910135327));
#105632=CARTESIAN_POINT('Ctrl Pts',(-16.6555831790833,18.8086411456773,
-12.3332796143443));
#105633=CARTESIAN_POINT('Ctrl Pts',(-16.6564405547861,18.8042373175098,
-12.3335527044166));
#105634=CARTESIAN_POINT('Ctrl Pts',(-16.6590085506938,18.7912669934161,
-12.3343598057923));
#105635=CARTESIAN_POINT('Ctrl Pts',(-16.6607581789969,18.7827084437987,
-12.3348959628262));
#105636=CARTESIAN_POINT('Ctrl Pts',(-16.6736571237646,18.721543140939,-12.3387522016628));
#105637=CARTESIAN_POINT('Ctrl Pts',(-16.6867534426695,18.6693716591661,
-12.3421709146376));
#105638=CARTESIAN_POINT('Ctrl Pts',(-16.7104391642818,18.5882347163738,
-12.3476350995392));
#105639=CARTESIAN_POINT('Ctrl Pts',(-16.7197005676377,18.558901282634,-12.3496416651875));
#105640=CARTESIAN_POINT('Ctrl Pts',(-16.7713011535742,18.4070729532009,
-12.3601590876147));
#105641=CARTESIAN_POINT('Ctrl Pts',(-16.82418860556,18.2884440129881,-12.3688059240255));
#105642=CARTESIAN_POINT('Ctrl Pts',(-16.9306717659915,18.0985923569696,
-12.3828985068889));
#105643=CARTESIAN_POINT('Ctrl Pts',(-16.9785032679527,18.0245438908122,
-12.388473936393));
#105644=CARTESIAN_POINT('Ctrl Pts',(-17.0429891587583,17.9371901485475,
-12.3951372929841));
#105645=CARTESIAN_POINT('Ctrl Pts',(-17.055402945988,17.9208755178247,-12.3963860190921));
#105646=CARTESIAN_POINT('Ctrl Pts',(-17.0735170210324,17.8977735459857,
-12.3981609332677));
#105647=CARTESIAN_POINT('Ctrl Pts',(-17.0790257002158,17.8908380729079,
-12.3986946660552));
#105648=CARTESIAN_POINT('Ctrl Pts',(-17.0886518177924,17.8788736556669,
-12.3996170229862));
#105649=CARTESIAN_POINT('Ctrl Pts',(-17.0927491582007,17.8738287642508,
-12.4000064453681));
#105650=CARTESIAN_POINT('Ctrl Pts',(-17.100672643188,17.8641641805943,-12.4007534761138));
#105651=CARTESIAN_POINT('Ctrl Pts',(-17.1044953118977,17.859541731485,-12.4011112196286));
#105652=CARTESIAN_POINT('Ctrl Pts',(-17.1145624057919,17.8474732077344,
-12.4020464554971));
#105653=CARTESIAN_POINT('Ctrl Pts',(-17.1208385912739,17.840053717704,-12.4026226469948));
#105654=CARTESIAN_POINT('Ctrl Pts',(-17.1428054609125,17.8144449636284,
-12.4046159558711));
#105655=CARTESIAN_POINT('Ctrl Pts',(-17.1587548347637,17.796479314563,-12.4060223845816));
#105656=CARTESIAN_POINT('Ctrl Pts',(-17.2751316001207,17.6698007100448,
-12.4160079827468));
#105657=CARTESIAN_POINT('Ctrl Pts',(-17.386410726083,17.5716092324639,-12.4240787171203));
#105658=CARTESIAN_POINT('Ctrl Pts',(-17.5447466168555,17.4589991622943,
-12.4346304835519));
#105659=CARTESIAN_POINT('Ctrl Pts',(-17.5833272620597,17.4334222395349,
-12.4371410213788));
#105660=CARTESIAN_POINT('Ctrl Pts',(-17.6834791700664,17.3716545246044,
-12.4435777414851));
#105661=CARTESIAN_POINT('Ctrl Pts',(-17.7460962079574,17.3372790125278,
-12.4475279674693));
#105662=CARTESIAN_POINT('Ctrl Pts',(-17.8405333843261,17.2914861123943,
-12.4535472390394));
#105663=CARTESIAN_POINT('Ctrl Pts',(-17.8710846401087,17.2775592965727,
-12.4555037594948));
#105664=CARTESIAN_POINT('Ctrl Pts',(-17.9086747925823,17.2614921765919,
-12.4579374025227));
#105665=CARTESIAN_POINT('Ctrl Pts',(-17.9154122191964,17.2586535929542,
-12.4583746100309));
#105666=CARTESIAN_POINT('Ctrl Pts',(-17.925974092016,17.2542679920748,-12.4590617844941));
#105667=CARTESIAN_POINT('Ctrl Pts',(-17.9297886608853,17.2526971275658,
-12.4593103307196));
#105668=CARTESIAN_POINT('Ctrl Pts',(-17.9369125936265,17.2497877702468,
-12.4597752262529));
#105669=CARTESIAN_POINT('Ctrl Pts',(-17.9402207598512,17.2484464947928,
-12.4599914043886));
#105670=CARTESIAN_POINT('Ctrl Pts',(-17.9477608880499,17.2454115800384,
-12.4604847862257));
#105671=CARTESIAN_POINT('Ctrl Pts',(-17.9519949205355,17.2437232445228,
-12.4607623038403));
#105672=CARTESIAN_POINT('Ctrl Pts',(-17.963017283664,17.2393692438376,-12.4614859101291));
#105673=CARTESIAN_POINT('Ctrl Pts',(-17.9698139289861,17.2367249855006,
-12.4619332341893));
#105674=CARTESIAN_POINT('Ctrl Pts',(-18.0131755332702,17.2201124589298,
-12.4647936639114));
#105675=CARTESIAN_POINT('Ctrl Pts',(-18.0501058423478,17.2071263895655,
-12.4672594017656));
#105676=CARTESIAN_POINT('Ctrl Pts',(-18.0991267188595,17.191401696334,-12.4705518240767));
#105677=CARTESIAN_POINT('Ctrl Pts',(-18.1109139992187,17.1877340223886,
-12.471344966723));
#105678=CARTESIAN_POINT('Ctrl Pts',(-18.1458487460221,17.1771981247549,
-12.4736987158397));
#105679=CARTESIAN_POINT('Ctrl Pts',(-18.1690820010302,17.1706226923207,
-12.4752680034453));
#105680=CARTESIAN_POINT('Ctrl Pts',(-18.3317803114042,17.1275679579354,
-12.486263746072));
#105681=CARTESIAN_POINT('Ctrl Pts',(-18.474555156648,17.1050172913893,-12.4959108700233));
#105682=CARTESIAN_POINT('Ctrl Pts',(-18.6802311390641,17.0937805087175,
-12.5092191237075));
#105683=CARTESIAN_POINT('Ctrl Pts',(-18.742071142451,17.0931129746865,-12.5131507151506));
#105684=CARTESIAN_POINT('Ctrl Pts',(-18.8410951749605,17.0963823391104,
-12.5193243378294));
#105685=CARTESIAN_POINT('Ctrl Pts',(-18.8782965770677,17.0985947351868,
-12.5216162848772));
#105686=CARTESIAN_POINT('Ctrl Pts',(-18.9265161335453,17.1027423009678,
-12.524553380184));
#105687=CARTESIAN_POINT('Ctrl Pts',(-18.9376025846519,17.1037840684572,
-12.5252263607198));
#105688=CARTESIAN_POINT('Ctrl Pts',(-18.9556144881182,17.1056200820621,
-12.5263161115541));
#105689=CARTESIAN_POINT('Ctrl Pts',(-18.9625450379386,17.1063611360517,
-12.5267345477325));
#105690=CARTESIAN_POINT('Ctrl Pts',(-18.9758627017549,17.1078516961695,
-12.527536971656));
#105691=CARTESIAN_POINT('Ctrl Pts',(-18.982250298083,17.1085961031914,-12.5279211153193));
#105692=CARTESIAN_POINT('Ctrl Pts',(-18.9968632870301,17.1103666193308,
-12.5287983086816));
#105693=CARTESIAN_POINT('Ctrl Pts',(-19.005086276883,17.1114119591885,-12.529290746441));
#105694=CARTESIAN_POINT('Ctrl Pts',(-19.0269054855044,17.1143160272117,
-12.5305944022915));
#105695=CARTESIAN_POINT('Ctrl Pts',(-19.0404902723101,17.1162587196999,
-12.5314029686364));
#105696=CARTESIAN_POINT('Ctrl Pts',(-19.1432879122264,17.1319807392357,
-12.5374998057136));
#105697=CARTESIAN_POINT('Ctrl Pts',(-19.2315620098317,17.151322211414,-12.5426055874753));
#105698=CARTESIAN_POINT('Ctrl Pts',(-19.4524107327221,17.2147454339367,
-12.5553255610993));
#105699=CARTESIAN_POINT('Ctrl Pts',(-19.5823414515173,17.2664020464035,
-12.5627450233497));
#105700=CARTESIAN_POINT('Ctrl Pts',(-19.7553604186876,17.3558533540198,
-12.5735037596431));
#105701=CARTESIAN_POINT('Ctrl Pts',(-19.8034593726833,17.3831592019586,
-12.5766018660388));
#105702=CARTESIAN_POINT('Ctrl Pts',(-19.8746319756805,17.4273355050485,
-12.581433751383));
#105703=CARTESIAN_POINT('Ctrl Pts',(-19.8985260758143,17.4428430009495,
-12.5831003971749));
#105704=CARTESIAN_POINT('Ctrl Pts',(-19.9278456879129,17.4627237955927,
-12.5852110176198));
#105705=CARTESIAN_POINT('Ctrl Pts',(-19.9335733773526,17.4666488533715,
-12.5856265097071));
#105706=CARTESIAN_POINT('Ctrl Pts',(-19.942606418798,17.4729045247935,-12.5862869921594));
#105707=CARTESIAN_POINT('Ctrl Pts',(-19.9459246375478,17.4752165950882,
-12.5865307376505));
#105708=CARTESIAN_POINT('Ctrl Pts',(-19.9521703955418,17.4795951575709,
-12.5869916929442));
#105709=CARTESIAN_POINT('Ctrl Pts',(-19.955099320414,17.4816595795131,-12.5872087621034));
#105710=CARTESIAN_POINT('Ctrl Pts',(-19.9617838702117,17.4863965628554,
-12.5877062306935));
#105711=CARTESIAN_POINT('Ctrl Pts',(-19.9655360125942,17.4890739574188,
-12.5879869595359));
#105712=CARTESIAN_POINT('Ctrl Pts',(-19.9754745481618,17.4962148412065,
-12.5887344477188));
#105713=CARTESIAN_POINT('Ctrl Pts',(-19.9816455446555,17.5006995043469,
-12.5892026121565));
#105714=CARTESIAN_POINT('Ctrl Pts',(-20.0247025244535,17.532347439808,-12.592496746876));
#105715=CARTESIAN_POINT('Ctrl Pts',(-20.0607197676149,17.560666277959,-12.5953947809447));
#105716=CARTESIAN_POINT('Ctrl Pts',(-20.1245701489341,17.6143106424667,
-12.6007562174839));
#105717=CARTESIAN_POINT('Ctrl Pts',(-20.1527028149936,17.6392543652428,
-12.6032035793863));
#105718=CARTESIAN_POINT('Ctrl Pts',(-20.275819313844,17.7544146700018,-12.6142536960959));
#105719=CARTESIAN_POINT('Ctrl Pts',(-20.362979256332,17.8525899411399,-12.6229968955414));
#105720=CARTESIAN_POINT('Ctrl Pts',(-20.4927972962823,18.0294209959865,
-12.6372013617079));
#105721=CARTESIAN_POINT('Ctrl Pts',(-20.5405828374066,18.1038601044472,
-12.6427967603634));
#105722=CARTESIAN_POINT('Ctrl Pts',(-20.5935715881277,18.1990196359036,
-12.6494812675744));
#105723=CARTESIAN_POINT('Ctrl Pts',(-20.6033012801272,18.2171068873108,
-12.6507323208643));
#105724=CARTESIAN_POINT('Ctrl Pts',(-20.6168513893215,18.2431992949443,
-12.652509930538));
#105725=CARTESIAN_POINT('Ctrl Pts',(-20.6208868700635,18.2510908885253,
-12.6530440631504));
#105726=CARTESIAN_POINT('Ctrl Pts',(-20.6277957964382,18.2648135838021,
-12.6539668888513));
#105727=CARTESIAN_POINT('Ctrl Pts',(-20.6306921431392,18.2706329607962,
-12.6543563824189));
#105728=CARTESIAN_POINT('Ctrl Pts',(-20.6362088781865,18.2818464365402,
-12.655103395696));
#105729=CARTESIAN_POINT('Ctrl Pts',(-20.6388332360891,18.2872385023335,
-12.6554610512908));
#105730=CARTESIAN_POINT('Ctrl Pts',(-20.6456466883697,18.3013900757899,
-12.6563957159273));
#105731=CARTESIAN_POINT('Ctrl Pts',(-20.6497985245005,18.3101674441554,
-12.656971427242));
#105732=CARTESIAN_POINT('Ctrl Pts',(-20.6639911334815,18.3407138870399,
-12.6589614020745));
#105733=CARTESIAN_POINT('Ctrl Pts',(-20.6737226592922,18.3626252198241,
-12.6603650251453));
#105734=CARTESIAN_POINT('Ctrl Pts',(-20.6971018560742,18.4177720291238,
-12.6638422012189));
#105735=CARTESIAN_POINT('Ctrl Pts',(-20.7102719365412,18.4511802539283,
-12.6658991156327));
#105736=CARTESIAN_POINT('Ctrl Pts',(-20.7225805288028,18.4848894846743,
-12.6679318969538));
#105737=CARTESIAN_POINT('',(-20.853822991173,19.2120774369757,-11.6890562790225));
#105738=CARTESIAN_POINT('Ctrl Pts',(-20.7242505411024,18.4842642021379,
-12.4443820858314));
#105739=CARTESIAN_POINT('Ctrl Pts',(-20.5136267642773,17.9235819449507,
-12.408272473254));
#105740=CARTESIAN_POINT('Ctrl Pts',(-19.5197099237742,16.8917269399042,
-12.329770925116));
#105741=CARTESIAN_POINT('Ctrl Pts',(-17.2597752565566,17.1878855805931,
-12.2088774414178));
#105742=CARTESIAN_POINT('Ctrl Pts',(-16.2349110453346,19.3555162442872,
-12.0817016347362));
#105743=CARTESIAN_POINT('Ctrl Pts',(-17.5028058390645,21.3905622235373,
-11.9545258280549));
#105744=CARTESIAN_POINT('Ctrl Pts',(-19.9002448589247,21.4259951415803,
-11.8273500213734));
#105745=CARTESIAN_POINT('Ctrl Pts',(-20.8239162970475,20.0366853799179,
-11.7388601716959));
#105746=CARTESIAN_POINT('Ctrl Pts',(-20.8542040955766,19.273466074897,-11.692762257579));
#105747=CARTESIAN_POINT('Ctrl Pts',(-20.853822991173,19.2120774369757,-11.6890562790225));
#105748=CARTESIAN_POINT('Ctrl Pts',(-20.8509997772511,19.2119711430765,
-11.6906773760522));
#105749=CARTESIAN_POINT('Ctrl Pts',(-20.8510795350122,19.038106790205,-11.6794937446562));
#105750=CARTESIAN_POINT('Ctrl Pts',(-20.829741896744,18.8648839271554,-11.6677631723301));
#105751=CARTESIAN_POINT('Ctrl Pts',(-20.7726123086137,18.637001790048,-11.6525929998784));
#105752=CARTESIAN_POINT('Ctrl Pts',(-20.7552164348725,18.5784659652781,
-11.648712755995));
#105753=CARTESIAN_POINT('Ctrl Pts',(-20.7311768486813,18.50876455386,-11.6441198123401));
#105754=CARTESIAN_POINT('Ctrl Pts',(-20.7269322965609,18.4968075654787,
-11.6433328539868));
#105755=CARTESIAN_POINT('Ctrl Pts',(-20.7225806143616,18.4848897189921,
-11.6425493859455));
#105756=CARTESIAN_POINT('Origin',(-18.734,19.211,0.));
#105757=CARTESIAN_POINT('',(-20.7225806140666,18.4848897181842,-10.844119113415));
#105758=CARTESIAN_POINT('',(-20.7225806135353,18.4848897167291,-11.0644159212905));
#105759=CARTESIAN_POINT('',(-20.7225806137986,18.4848897174502,0.));
#105760=CARTESIAN_POINT('Ctrl Pts',(-20.7225806135353,18.4848897167291,
-11.0644159212905));
#105761=CARTESIAN_POINT('Ctrl Pts',(-20.7579845105336,18.5818495103536,
-11.0708124284518));
#105762=CARTESIAN_POINT('Ctrl Pts',(-20.7862468955592,18.6812615260696,
-11.0775606980553));
#105763=CARTESIAN_POINT('Ctrl Pts',(-20.8362075141281,18.9228812641263,
-11.0938351530036));
#105764=CARTESIAN_POINT('Ctrl Pts',(-20.8509047690515,19.066044097594,-11.1033537530625));
#105765=CARTESIAN_POINT('Ctrl Pts',(-20.8510404641561,19.2715966101103,
-11.1164063739387));
#105766=CARTESIAN_POINT('Ctrl Pts',(-20.8483582574222,19.3335670541364,
-11.1202674161294));
#105767=CARTESIAN_POINT('Ctrl Pts',(-20.8418780039395,19.4077067100225,
-11.1248002039059));
#105768=CARTESIAN_POINT('Ctrl Pts',(-20.8406878629333,19.4200680935513,
-11.1255531154824));
#105769=CARTESIAN_POINT('Ctrl Pts',(-20.8385539134696,19.4403590526985,
-11.1267844866857));
#105770=CARTESIAN_POINT('Ctrl Pts',(-20.8376739011466,19.4482949011569,
-11.1272649420936));
#105771=CARTESIAN_POINT('Ctrl Pts',(-20.8360103028606,19.4625598420287,
-11.1281265864217));
#105772=CARTESIAN_POINT('Ctrl Pts',(-20.8352429787453,19.4688906999214,
-11.1285082828655));
#105773=CARTESIAN_POINT('Ctrl Pts',(-20.8335469912837,19.4823732454618,
-11.129319698516));
#105774=CARTESIAN_POINT('Ctrl Pts',(-20.8326103655088,19.4895238638156,
-11.1297491613722));
#105775=CARTESIAN_POINT('Ctrl Pts',(-20.8299874443797,19.5087836537127,
-11.1309035996037));
#105776=CARTESIAN_POINT('Ctrl Pts',(-20.8282327450459,19.5208833497365,
-11.1316264082981));
#105777=CARTESIAN_POINT('Ctrl Pts',(-20.8189028588071,19.5815155976498,
-11.1352369428666));
#105778=CARTESIAN_POINT('Ctrl Pts',(-20.8097446645727,19.6297915688479,
-11.1380741497991));
#105779=CARTESIAN_POINT('Ctrl Pts',(-20.7784289229906,19.7683456731649,
-11.1461497914733));
#105780=CARTESIAN_POINT('Ctrl Pts',(-20.7519966827993,19.8575409818251,
-11.1512603952119));
#105781=CARTESIAN_POINT('Ctrl Pts',(-20.66234994469,20.1001681817574,-11.1653489191763));
#105782=CARTESIAN_POINT('Ctrl Pts',(-20.5868669495829,20.2483141193899,
-11.1741493678622));
#105783=CARTESIAN_POINT('Ctrl Pts',(-20.4871421973997,20.3977505899914,
-11.1847107456619));
#105784=CARTESIAN_POINT('Ctrl Pts',(-20.4792655410229,20.4093040912681,
-11.1855394060308));
#105785=CARTESIAN_POINT('Ctrl Pts',(-20.4681194497217,20.4253101871166,
-11.1867057080819));
#105786=CARTESIAN_POINT('Ctrl Pts',(-20.4649459694673,20.4298295802376,
-11.1870370775382));
#105787=CARTESIAN_POINT('Ctrl Pts',(-20.4598136883828,20.4370780552825,
-11.1875719580491));
#105788=CARTESIAN_POINT('Ctrl Pts',(-20.4578659860817,20.4398150171287,
-11.1877747111508));
#105789=CARTESIAN_POINT('Ctrl Pts',(-20.453774817535,20.4455351639029,-11.1882001338125));
#105790=CARTESIAN_POINT('Ctrl Pts',(-20.4516300989897,20.4485174084696,
-11.1884228927116));
#105791=CARTESIAN_POINT('Ctrl Pts',(-20.4464076165461,20.4557395730299,
-11.1889646604425));
#105792=CARTESIAN_POINT('Ctrl Pts',(-20.443321864483,20.4599736635019,-11.1892842171977));
#105793=CARTESIAN_POINT('Ctrl Pts',(-20.4323912729261,20.4748556101276,
-11.1904141130635));
#105794=CARTESIAN_POINT('Ctrl Pts',(-20.4244625874357,20.4854411086334,
-11.1912299895));
#105795=CARTESIAN_POINT('Ctrl Pts',(-20.3764349025933,20.5483255775225,
-11.1961467361627));
#105796=CARTESIAN_POINT('Ctrl Pts',(-20.3340141770669,20.5987986407266,
-11.2003844694808));
#105797=CARTESIAN_POINT('Ctrl Pts',(-20.2240817826416,20.7178479439201,
-11.2109621072753));
#105798=CARTESIAN_POINT('Ctrl Pts',(-20.1541137643016,20.7839625451605,
-11.2173577785994));
#105799=CARTESIAN_POINT('Ctrl Pts',(-19.9712621247926,20.934565486735,-11.2329413186586));
#105800=CARTESIAN_POINT('Ctrl Pts',(-19.8539618969555,21.0129972743543,
-11.2419898570745));
#105801=CARTESIAN_POINT('Ctrl Pts',(-19.717114103807,21.0859346183671,-11.2514585061595));
#105802=CARTESIAN_POINT('Ctrl Pts',(-19.7044367168009,21.0925275067495,
-11.252326436666));
#105803=CARTESIAN_POINT('Ctrl Pts',(-19.6841535555004,21.1028162426984,
-11.253700687019));
#105804=CARTESIAN_POINT('Ctrl Pts',(-19.6765908815097,21.1065956606042,
-11.2542099345473));
#105805=CARTESIAN_POINT('Ctrl Pts',(-19.6632128769917,21.1131814103799,
-11.2551052974857));
#105806=CARTESIAN_POINT('Ctrl Pts',(-19.6574070058504,21.1160066119941,
-11.2554920689526));
#105807=CARTESIAN_POINT('Ctrl Pts',(-19.6453717560817,21.1217951503559,
-11.2562901406439));
#105808=CARTESIAN_POINT('Ctrl Pts',(-19.6391406299403,21.1247546933111,
-11.2567013054508));
#105809=CARTESIAN_POINT('Ctrl Pts',(-19.6231088252015,21.1322733622453,
-11.257754043659));
#105810=CARTESIAN_POINT('Ctrl Pts',(-19.6132874172106,21.1367880153378,
-11.2583940755956));
#105811=CARTESIAN_POINT('Ctrl Pts',(-19.5721500245015,21.1553175190691,
-11.2610549656036));
#105812=CARTESIAN_POINT('Ctrl Pts',(-19.5405292286959,21.1686457489669,
-11.2630522898664));
#105813=CARTESIAN_POINT('Ctrl Pts',(-19.4573061357852,21.2013654524187,
-11.2681969868866));
#105814=CARTESIAN_POINT('Ctrl Pts',(-19.4052450006245,21.2195211462679,
-11.2713049582114));
#105815=CARTESIAN_POINT('Ctrl Pts',(-19.2479504672115,21.2675752924697,
-11.2804500881202));
#105816=CARTESIAN_POINT('Ctrl Pts',(-19.141048083626,21.2913749077612,-11.2863385197153));
#105817=CARTESIAN_POINT('Ctrl Pts',(-18.9869092014435,21.3133494929698,
-11.2948153695867));
#105818=CARTESIAN_POINT('Ctrl Pts',(-18.9408313281924,21.3183815524446,
-11.2973493293416));
#105819=CARTESIAN_POINT('Ctrl Pts',(-18.8732956181031,21.3235206250554,
-11.3011064779075));
#105820=CARTESIAN_POINT('Ctrl Pts',(-18.8519413958002,21.3248203435619,
-11.3023007734537));
#105821=CARTESIAN_POINT('Ctrl Pts',(-18.7787711723302,21.3281616443893,
-11.3064252218375));
#105822=CARTESIAN_POINT('Ctrl Pts',(-18.726905702043,21.3286228685763,-11.3094038698376));
#105823=CARTESIAN_POINT('Ctrl Pts',(-18.6664284876887,21.3269390361204,
-11.3129946257956));
#105824=CARTESIAN_POINT('Ctrl Pts',(-18.6577782873495,21.3266450927753,
-11.3135110326991));
#105825=CARTESIAN_POINT('Ctrl Pts',(-18.6446646719969,21.3261189501094,
-11.3142984925047));
#105826=CARTESIAN_POINT('Ctrl Pts',(-18.6401996689471,21.3259256419538,
-11.3145674193035));
#105827=CARTESIAN_POINT('Ctrl Pts',(-18.6321761092844,21.32555281109,-11.3150521828745));
#105828=CARTESIAN_POINT('Ctrl Pts',(-18.628617367591,21.3253784420222,-11.3152677282955));
#105829=CARTESIAN_POINT('Ctrl Pts',(-18.6208738442635,21.3249794311378,
-11.3157379127352));
#105830=CARTESIAN_POINT('Ctrl Pts',(-18.6166893381185,21.3247513501573,
-11.3159927369557));
#105831=CARTESIAN_POINT('Ctrl Pts',(-18.6049073174612,21.3240740648805,
-11.3167122654164));
#105832=CARTESIAN_POINT('Ctrl Pts',(-18.5973115984563,21.323596317615,-11.3171785233143));
#105833=CARTESIAN_POINT('Ctrl Pts',(-18.5512927044935,21.3204526531747,
-11.3200171573825));
#105834=CARTESIAN_POINT('Ctrl Pts',(-18.5129481501408,21.3167796894321,
-11.322440642795));
#105835=CARTESIAN_POINT('Ctrl Pts',(-18.3856325083811,21.3010688941811,
-11.3306356250005));
#105836=CARTESIAN_POINT('Ctrl Pts',(-18.2973319041579,21.2844191284673,
-11.3365582415861));
#105837=CARTESIAN_POINT('Ctrl Pts',(-18.0441487550144,21.2197859751892,
-11.3538252853405));
#105838=CARTESIAN_POINT('Ctrl Pts',(-17.8836768076623,21.157301178375,-11.3650716755558));
#105839=CARTESIAN_POINT('Ctrl Pts',(-17.7119976962816,21.0651146703995,
-11.3770690601322));
#105840=CARTESIAN_POINT('Ctrl Pts',(-17.6916893340496,21.0537746642382,
-11.3784891042215));
#105841=CARTESIAN_POINT('Ctrl Pts',(-17.6632763498872,21.0372890885449,
-11.3804777712047));
#105842=CARTESIAN_POINT('Ctrl Pts',(-17.6550140828128,21.0324198761118,
-11.381056296067));
#105843=CARTESIAN_POINT('Ctrl Pts',(-17.6416584027079,21.0244261862462,
-11.3819919316247));
#105844=CARTESIAN_POINT('Ctrl Pts',(-17.6365446974493,21.0213360346021,
-11.3823502864271));
#105845=CARTESIAN_POINT('Ctrl Pts',(-17.6258801442078,21.0148297772442,
-11.3830978964969));
#105846=CARTESIAN_POINT('Ctrl Pts',(-17.6203318449393,21.0114095983811,
-11.3834869973548));
#105847=CARTESIAN_POINT('Ctrl Pts',(-17.6071923222302,21.0032259266913,
-11.3844088800682));
#105848=CARTESIAN_POINT('Ctrl Pts',(-17.5996153382607,20.9984397214894,
-11.3849408172334));
#105849=CARTESIAN_POINT('Ctrl Pts',(-17.574294126043,20.9822190376323,-11.386719781641));
#105850=CARTESIAN_POINT('Ctrl Pts',(-17.5566902158126,20.9705670811004,
-11.387958712242));
#105851=CARTESIAN_POINT('Ctrl Pts',(-17.4624601024923,20.9061491620252,
-11.3946072690356));
#105852=CARTESIAN_POINT('Ctrl Pts',(-17.3891969459869,20.8486361132048,
-11.3998312982591));
#105853=CARTESIAN_POINT('Ctrl Pts',(-17.2047827469816,20.6831179258877,
-11.4134775863346));
#105854=CARTESIAN_POINT('Ctrl Pts',(-17.1013074763857,20.5674458252306,
-11.4216609279055));
#105855=CARTESIAN_POINT('Ctrl Pts',(-16.9802032397533,20.3979122248355,
-11.433375191727));
#105856=CARTESIAN_POINT('Ctrl Pts',(-16.9507093259367,20.3531195403558,
-11.4364511156338));
#105857=CARTESIAN_POINT('Ctrl Pts',(-16.9184242281447,20.2997837226892,
-11.4401507752034));
#105858=CARTESIAN_POINT('Ctrl Pts',(-16.9139450443887,20.2922794878011,
-11.440672140623));
#105859=CARTESIAN_POINT('Ctrl Pts',(-16.9072365356623,20.2808805455965,
-11.4414656846782));
#105860=CARTESIAN_POINT('Ctrl Pts',(-16.9049728563827,20.2770060241592,
-11.4417356876353));
#105861=CARTESIAN_POINT('Ctrl Pts',(-16.9009333090442,20.2700411750234,
-11.4422215935871));
#105862=CARTESIAN_POINT('Ctrl Pts',(-16.8991529127134,20.2669535358476,
-11.4424371990941));
#105863=CARTESIAN_POINT('Ctrl Pts',(-16.8953030730426,20.2602378451347,
-11.4429065810143));
#105864=CARTESIAN_POINT('Ctrl Pts',(-16.8932365938309,20.2566082089763,
-11.4431605375263));
#105865=CARTESIAN_POINT('Ctrl Pts',(-16.8874667558539,20.2464037482004,
-11.4438752201855));
#105866=CARTESIAN_POINT('Ctrl Pts',(-16.8837878339844,20.2398152799768,
-11.4443374673691));
#105867=CARTESIAN_POINT('Ctrl Pts',(-16.862096123084,20.2004756093816,-11.4471017330519));
#105868=CARTESIAN_POINT('Ctrl Pts',(-16.844919248195,20.1672738219225,-11.449451863414));
#105869=CARTESIAN_POINT('Ctrl Pts',(-16.7914740506213,20.0569023890397,
-11.457278254883));
#105870=CARTESIAN_POINT('Ctrl Pts',(-16.7589884595079,19.9779976928646,
-11.4628922166034));
#105871=CARTESIAN_POINT('Ctrl Pts',(-16.673653546085,19.7290072475013,-11.4802802430761));
#105872=CARTESIAN_POINT('Ctrl Pts',(-16.6374025011106,19.5540195074303,
-11.4919745855397));
#105873=CARTESIAN_POINT('Ctrl Pts',(-16.6216992387344,19.3538082222448,
-11.5043334514449));
#105874=CARTESIAN_POINT('Ctrl Pts',(-16.6202838466278,19.3310532429137,
-11.5057249444752));
#105875=CARTESIAN_POINT('Ctrl Pts',(-16.6187990464069,19.2987749728946,
-11.5076808587237));
#105876=CARTESIAN_POINT('Ctrl Pts',(-16.6184259253278,19.2892678678961,
-11.5082547466318));
#105877=CARTESIAN_POINT('Ctrl Pts',(-16.6179232947684,19.2738005683485,
-11.5091849231686));
#105878=CARTESIAN_POINT('Ctrl Pts',(-16.61775484906,19.2678418513155,-11.5095424274324));
#105879=CARTESIAN_POINT('Ctrl Pts',(-16.617454632156,19.2553547260921,-11.5102898801202));
#105880=CARTESIAN_POINT('Ctrl Pts',(-16.6173278921667,19.2488262509701,
-11.5106796670301));
#105881=CARTESIAN_POINT('Ctrl Pts',(-16.6170978946007,19.2332705124533,
-11.5116061146544));
#105882=CARTESIAN_POINT('Ctrl Pts',(-16.617022171013,19.2242429223034,-11.5121419078479));
#105883=CARTESIAN_POINT('Ctrl Pts',(-16.6169613931839,19.1937172004032,
-11.5139475471835));
#105884=CARTESIAN_POINT('Ctrl Pts',(-16.6172460522855,19.1722194270122,
-11.515208956021));
#105885=CARTESIAN_POINT('Ctrl Pts',(-16.6229706616906,18.9712254259447,
-11.5269162695944));
#105886=CARTESIAN_POINT('Ctrl Pts',(-16.6508996755496,18.7931044056527,
-11.53656416354));
#105887=CARTESIAN_POINT('Ctrl Pts',(-16.734548283313,18.50504787237,-11.5528890786301));
#105888=CARTESIAN_POINT('Ctrl Pts',(-16.7779045786298,18.3925515737823,
-11.5594929098358));
#105889=CARTESIAN_POINT('Ctrl Pts',(-16.8347306148411,18.2758235145013,
-11.5671871224211));
#105890=CARTESIAN_POINT('Ctrl Pts',(-16.8389463840805,18.2673098805152,
-11.5677534037208));
#105891=CARTESIAN_POINT('Ctrl Pts',(-16.8452798834752,18.2547331377544,
-11.5685979463252));
#105892=CARTESIAN_POINT('Ctrl Pts',(-16.8473537985084,18.2506479292017,
-11.568873533089));
#105893=CARTESIAN_POINT('Ctrl Pts',(-16.8510681791836,18.2433897908696,
-11.5693654680895));
#105894=CARTESIAN_POINT('Ctrl Pts',(-16.8527034300416,18.2402142490287,
-11.5695814871177));
#105895=CARTESIAN_POINT('Ctrl Pts',(-16.8562374571197,18.2333938819136,
-11.5700471661826));
#105896=CARTESIAN_POINT('Ctrl Pts',(-16.8581387844127,18.2297504961754,
-11.5702969816558));
#105897=CARTESIAN_POINT('Ctrl Pts',(-16.8634187448824,18.2197042925756,
-11.5709886828184));
#105898=CARTESIAN_POINT('Ctrl Pts',(-16.8668195948237,18.2133133043919,
-11.5714319390947));
#105899=CARTESIAN_POINT('Ctrl Pts',(-16.8856710911908,18.178320955691,-11.573876105825));
#105900=CARTESIAN_POINT('Ctrl Pts',(-16.9017452797992,18.1500626147046,
-11.5759132922613));
#105901=CARTESIAN_POINT('Ctrl Pts',(-17.002156459529,17.9826322821542,-11.5883186817831));
#105902=CARTESIAN_POINT('Ctrl Pts',(-17.1016589033143,17.8531959753851,
-11.599277255974));
#105903=CARTESIAN_POINT('Ctrl Pts',(-17.2963410340352,17.6526477544578,
-11.6175341145785));
#105904=CARTESIAN_POINT('Ctrl Pts',(-17.3844807291122,17.5757230941183,
-11.6249726280474));
#105905=CARTESIAN_POINT('Ctrl Pts',(-17.4900556557493,17.4979628239627,
-11.6329791293076));
#105906=CARTESIAN_POINT('Ctrl Pts',(-17.5016671086332,17.4895908218166,
-11.6338486392411));
#105907=CARTESIAN_POINT('Ctrl Pts',(-17.5202763420332,17.4764581345465,
-11.6352249096113));
#105908=CARTESIAN_POINT('Ctrl Pts',(-17.5272191397605,17.4716206395595,
-11.6357346111356));
#105909=CARTESIAN_POINT('Ctrl Pts',(-17.5395114379058,17.4631648305526,
-11.6366305022658));
#105910=CARTESIAN_POINT('Ctrl Pts',(-17.5448488054406,17.4595291488458,
-11.6370173503646));
#105911=CARTESIAN_POINT('Ctrl Pts',(-17.5559191274432,17.4520622522175,
-11.6378153218571));
#105912=CARTESIAN_POINT('Ctrl Pts',(-17.5616543368674,17.448234504898,-11.6382263111067));
#105913=CARTESIAN_POINT('Ctrl Pts',(-17.5764165323491,17.438485950845,-11.6392780656892));
#105914=CARTESIAN_POINT('Ctrl Pts',(-17.5854703612653,17.4326060013278,
-11.639917295209));
#105915=CARTESIAN_POINT('Ctrl Pts',(-17.6233835937971,17.4083938015694,
-11.6425703968292));
#105916=CARTESIAN_POINT('Ctrl Pts',(-17.6526409352452,17.3906921479872,
-11.6445609105989));
#105917=CARTESIAN_POINT('Ctrl Pts',(-17.7299177863768,17.3464581417023,
-11.64968411544));
#105918=CARTESIAN_POINT('Ctrl Pts',(-17.7785631999672,17.3210691568222,
-11.6527778353638));
#105919=CARTESIAN_POINT('Ctrl Pts',(-17.9986788056892,17.2168604124533,
-11.6663221766345));
#105920=CARTESIAN_POINT('Ctrl Pts',(-18.1792199646723,17.1592945482625,
-11.6761688900735));
#105921=CARTESIAN_POINT('Ctrl Pts',(-18.4061017136453,17.119130997804,-11.6892631781547));
#105922=CARTESIAN_POINT('Ctrl Pts',(-18.4474294347507,17.1130700683978,
-11.6916799805745));
#105923=CARTESIAN_POINT('Ctrl Pts',(-18.4962811643947,17.1073760113794,
-11.694602067743));
#105924=CARTESIAN_POINT('Ctrl Pts',(-18.5036605627018,17.1065552109255,
-11.695045217215));
#105925=CARTESIAN_POINT('Ctrl Pts',(-18.5156165850949,17.1052889972477,
-11.6957662516826));
#105926=CARTESIAN_POINT('Ctrl Pts',(-18.5201906832431,17.1048196377873,
-11.6960428244561));
#105927=CARTESIAN_POINT('Ctrl Pts',(-18.5283222704429,17.1040119977157,
-11.69653584019));
#105928=CARTESIAN_POINT('Ctrl Pts',(-18.5318791236986,17.1036678189359,
-11.6967519483542));
#105929=CARTESIAN_POINT('Ctrl Pts',(-18.5395176016138,17.1029481987413,
-11.6972170467616));
#105930=CARTESIAN_POINT('Ctrl Pts',(-18.5435993894904,17.1025756103358,
-11.6974661883741));
#105931=CARTESIAN_POINT('Ctrl Pts',(-18.554844328683,17.1015820845437,-11.6981541704597));
#105932=CARTESIAN_POINT('Ctrl Pts',(-18.5620095234353,17.100985789345,-11.6985943578276));
#105933=CARTESIAN_POINT('Ctrl Pts',(-18.6008731439588,17.0979507859534,
-11.7009912097525));
#105934=CARTESIAN_POINT('Ctrl Pts',(-18.6326186018115,17.0961900083692,
-11.7029825472233));
#105935=CARTESIAN_POINT('Ctrl Pts',(-18.8276392870077,17.0897739414869,
-11.7153728631945));
#105936=CARTESIAN_POINT('Ctrl Pts',(-18.9909572686806,17.1033138040003,
-11.7263739028625));
#105937=CARTESIAN_POINT('Ctrl Pts',(-19.2657918897069,17.158544528777,-11.7446861638805));
#105938=CARTESIAN_POINT('Ctrl Pts',(-19.3783966820372,17.1910651417365,
-11.7521391043154));
#105939=CARTESIAN_POINT('Ctrl Pts',(-19.5011180995793,17.2378240377561,
-11.7601580957281));
#105940=CARTESIAN_POINT('Ctrl Pts',(-19.5144314680354,17.2430517547101,
-11.7610268712044));
#105941=CARTESIAN_POINT('Ctrl Pts',(-19.5355324265156,17.251585211936,-11.7624022022785));
#105942=CARTESIAN_POINT('Ctrl Pts',(-19.5433547676538,17.2548033315233,
-11.7629116927266));
#105943=CARTESIAN_POINT('Ctrl Pts',(-19.5571145917463,17.2605608017561,
-11.7638073382533));
#105944=CARTESIAN_POINT('Ctrl Pts',(-19.5630600972131,17.2630805833315,
-11.7641941506921));
#105945=CARTESIAN_POINT('Ctrl Pts',(-19.5744693055324,17.2679776511708,
-11.7649361022921));
#105946=CARTESIAN_POINT('Ctrl Pts',(-19.5799346755131,17.270350874714,-11.7652913752427));
#105947=CARTESIAN_POINT('Ctrl Pts',(-19.5943386932351,17.2766779319188,
-11.7662273577707));
#105948=CARTESIAN_POINT('Ctrl Pts',(-19.6032601719841,17.2806706787676,
-11.7668067320043));
#105949=CARTESIAN_POINT('Ctrl Pts',(-19.6362975564567,17.2957318233745,
-11.7689512222639));
#105950=CARTESIAN_POINT('Ctrl Pts',(-19.6602329958321,17.3071918166191,
-11.7705028524968));
#105951=CARTESIAN_POINT('Ctrl Pts',(-19.719048608807,17.3367238841889,-11.774315361069));
#105952=CARTESIAN_POINT('Ctrl Pts',(-19.7536537925293,17.3553227311087,
-11.7765581797086));
#105953=CARTESIAN_POINT('Ctrl Pts',(-19.881612670487,17.4287562809325,-11.784882087309));
#105954=CARTESIAN_POINT('Ctrl Pts',(-19.9712357075821,17.4897628056551,
-11.7907658645788));
#105955=CARTESIAN_POINT('Ctrl Pts',(-20.162193736129,17.6424009371761,-11.8040415330628));
#105956=CARTESIAN_POINT('Ctrl Pts',(-20.2601157999815,17.7375005398172,
-11.8113988535014));
#105957=CARTESIAN_POINT('Ctrl Pts',(-20.3583117961853,17.8532283653158,
-11.8202986991472));
#105958=CARTESIAN_POINT('Ctrl Pts',(-20.3682779988764,17.8652407297263,
-11.8212220846294));
#105959=CARTESIAN_POINT('Ctrl Pts',(-20.381750003524,17.8818490267196,-11.8224999396963));
#105960=CARTESIAN_POINT('Ctrl Pts',(-20.3853714371822,17.886351081017,-11.8228464484126));
#105961=CARTESIAN_POINT('Ctrl Pts',(-20.3910999480515,17.8935325881788,
-11.823399473813));
#105962=CARTESIAN_POINT('Ctrl Pts',(-20.3932190925738,17.8962024408672,
-11.8236051336071));
#105963=CARTESIAN_POINT('Ctrl Pts',(-20.3975851129308,17.9017304366302,
-11.8240311140067));
#105964=CARTESIAN_POINT('Ctrl Pts',(-20.3998310708248,17.9045892452111,
-11.8242514995298));
#105965=CARTESIAN_POINT('Ctrl Pts',(-20.4051695365946,17.9114205585473,
-11.8247783135232));
#105966=CARTESIAN_POINT('Ctrl Pts',(-20.408255250054,17.9153983246562,-11.8250852187671));
#105967=CARTESIAN_POINT('Ctrl Pts',(-20.418634169762,17.9288766958081,-11.8261255400785));
#105968=CARTESIAN_POINT('Ctrl Pts',(-20.4258607732686,17.9384279738483,
-11.826863410319));
#105969=CARTESIAN_POINT('Ctrl Pts',(-20.5082141624011,18.0492144273899,
-11.8354246480051));
#105970=CARTESIAN_POINT('Ctrl Pts',(-20.5742271637865,18.1568942444952,
-11.8437557121081));
#105971=CARTESIAN_POINT('Ctrl Pts',(-20.6639654874019,18.3376911509954,
-11.8570944299295));
#105972=CARTESIAN_POINT('Ctrl Pts',(-20.6939974412518,18.4073544815339,
-11.8620973608283));
#105973=CARTESIAN_POINT('Ctrl Pts',(-20.721016234076,18.4806160848838,-11.8671696308045));
#105974=CARTESIAN_POINT('Ctrl Pts',(-20.7218001501807,18.4827522806762,
-11.8673173710366));
#105975=CARTESIAN_POINT('Ctrl Pts',(-20.7225806137507,18.4848897173191,
-11.8674650369494));
#105976=CARTESIAN_POINT('Ctrl Pts',(-20.7225806143616,18.4848897189921,
-11.6425493859455));
#105977=CARTESIAN_POINT('Ctrl Pts',(-20.7142679983043,18.4621241590236,
-11.6410527994022));
#105978=CARTESIAN_POINT('Ctrl Pts',(-20.7055644761456,18.4395014220629,
-11.6395689721133));
#105979=CARTESIAN_POINT('Ctrl Pts',(-20.6923109675864,18.4067423615176,
-11.6374245029276));
#105980=CARTESIAN_POINT('Ctrl Pts',(-20.6880673194941,18.3964859650925,
-11.63675370293));
#105981=CARTESIAN_POINT('Ctrl Pts',(-20.6810308679606,18.3798512349006,
-11.6356666001178));
#105982=CARTESIAN_POINT('Ctrl Pts',(-20.6782869568271,18.3734525674138,
-11.6352486465248));
#105983=CARTESIAN_POINT('Ctrl Pts',(-20.6729468957414,18.3611674735963,
-11.6344465570414));
#105984=CARTESIAN_POINT('Ctrl Pts',(-20.6703553845417,18.3552791263467,
-11.6340622683996));
#105985=CARTESIAN_POINT('Ctrl Pts',(-20.6643565558064,18.3418155784917,
-11.6331839240812));
#105986=CARTESIAN_POINT('Ctrl Pts',(-20.6609314031985,18.3342484037618,
-11.6326904859046));
#105987=CARTESIAN_POINT('Ctrl Pts',(-20.6517054394834,18.3141807586619,
-11.6313824212375));
#105988=CARTESIAN_POINT('Ctrl Pts',(-20.6458268972398,18.3017163079416,
-11.630570475544));
#105989=CARTESIAN_POINT('Ctrl Pts',(-20.5995489628504,18.2060249935389,
-11.6243392030782));
#105990=CARTESIAN_POINT('Ctrl Pts',(-20.5538524598522,18.1254642945199,
-11.619112129004));
#105991=CARTESIAN_POINT('Ctrl Pts',(-20.4258214013433,17.9306935849389,
-11.6062233157348));
#105992=CARTESIAN_POINT('Ctrl Pts',(-20.3371158370147,17.8212296950832,
-11.5987519188402));
#105993=CARTESIAN_POINT('Ctrl Pts',(-20.2010309774874,17.6838122192984,
-11.5880489838806));
#105994=CARTESIAN_POINT('Ctrl Pts',(-20.162450153694,17.6476664452851,-11.5850813872512));
#105995=CARTESIAN_POINT('Ctrl Pts',(-20.108701657067,17.6009622883346,-11.5809700625467));
#105996=CARTESIAN_POINT('Ctrl Pts',(-20.0946874260822,17.5891011865518,
-11.5799000500308));
#105997=CARTESIAN_POINT('Ctrl Pts',(-20.0737585435042,17.5718499606658,
-11.5783019343463));
#105998=CARTESIAN_POINT('Ctrl Pts',(-20.0669614688815,17.5663178048296,
-11.5777828900162));
#105999=CARTESIAN_POINT('Ctrl Pts',(-20.0546537165162,17.5564269053892,
-11.5768425879283));
#106000=CARTESIAN_POINT('Ctrl Pts',(-20.049155276356,17.5520530568212,-11.5764223531706));
#106001=CARTESIAN_POINT('Ctrl Pts',(-20.0404396658009,17.5451906044537,
-11.5757558051433));
#106002=CARTESIAN_POINT('Ctrl Pts',(-20.0372368644139,17.5426837178577,
-11.5755107717217));
#106003=CARTESIAN_POINT('Ctrl Pts',(-20.034017555783,17.5401788381769,-11.5752643616912));
#106004=CARTESIAN_POINT('Ctrl Pts',(-20.0340082213093,17.5401715753351,
-11.5752636472176));
#106005=CARTESIAN_POINT('Ctrl Pts',(-20.0339895166574,17.5401570221227,
-11.5752622155356));
#106006=CARTESIAN_POINT('Ctrl Pts',(-20.0339801462261,17.5401497315562,
-11.5752614983078));
#106007=CARTESIAN_POINT('Ctrl Pts',(-20.0339613686576,17.5401351221179,
-11.5752600610408));
#106008=CARTESIAN_POINT('Ctrl Pts',(-20.0339519622102,17.5401278037839,
-11.5752593410543));
#106009=CARTESIAN_POINT('Ctrl Pts',(-20.0339331125487,17.5401131387666,
-11.5752578982653));
#106010=CARTESIAN_POINT('Ctrl Pts',(-20.0339236691864,17.5401057919688,
-11.5752571754514));
#106011=CARTESIAN_POINT('Ctrl Pts',(-20.0339040666131,17.5400905417203,
-11.575255675029));
#106012=CARTESIAN_POINT('Ctrl Pts',(-20.0338939075657,17.540082638417,-11.5752548974329));
#106013=CARTESIAN_POINT('Ctrl Pts',(-20.0338734124997,17.5400666944345,
-11.5752533286926));
#106014=CARTESIAN_POINT('Ctrl Pts',(-20.0338630762897,17.5400586536116,
-11.5752525375338));
#106015=CARTESIAN_POINT('Ctrl Pts',(-20.0338422231017,17.540042431652,-11.5752509413773));
#106016=CARTESIAN_POINT('Ctrl Pts',(-20.0338317061711,17.5400342505576,
-11.5752501363832));
#106017=CARTESIAN_POINT('Ctrl Pts',(-20.0338104872993,17.5400177447709,
-11.5752485122314));
#106018=CARTESIAN_POINT('Ctrl Pts',(-20.0337997858628,17.5400094204769,
-11.5752476931123));
#106019=CARTESIAN_POINT('Ctrl Pts',(-20.0337781941368,17.5399926253195,
-11.5752460404161));
#106020=CARTESIAN_POINT('Ctrl Pts',(-20.0337673039442,17.5399841545371,
-11.5752452068464));
#106021=CARTESIAN_POINT('Ctrl Pts',(-20.03374533129,17.5399670637635,-11.5752435249875));
#106022=CARTESIAN_POINT('Ctrl Pts',(-20.0337342481511,17.5399584432516,
-11.5752426766464));
#106023=CARTESIAN_POINT('Ctrl Pts',(-20.0337118851474,17.5399410495704,
-11.5752409649035));
#106024=CARTESIAN_POINT('Ctrl Pts',(-20.0337006054112,17.5399322765076,
-11.5752401015114));
#106025=CARTESIAN_POINT('Ctrl Pts',(-20.0336778445948,17.5399145741522,
-11.5752383593127));
#106026=CARTESIAN_POINT('Ctrl Pts',(-20.0336663637293,17.5399056450331,
-11.5752374805226));
#106027=CARTESIAN_POINT('Ctrl Pts',(-20.0336431964986,17.5398876273529,
-11.5752357072096));
#106028=CARTESIAN_POINT('Ctrl Pts',(-20.0336315099244,17.5398785386362,
-11.5752348126707));
#106029=CARTESIAN_POINT('Ctrl Pts',(-20.0336079267838,17.5398601982874,
-11.5752330075162));
#106030=CARTESIAN_POINT('Ctrl Pts',(-20.0335960301635,17.5398509466207,
-11.5752320968964));
#106031=CARTESIAN_POINT('Ctrl Pts',(-20.0335720219904,17.5398322765518,
-11.5752302592018));
#106032=CARTESIAN_POINT('Ctrl Pts',(-20.0335599107319,17.5398228583858,
-11.5752293321494));
#106033=CARTESIAN_POINT('Ctrl Pts',(-20.0335354687951,17.5398038518512,
-11.575227461246));
#106034=CARTESIAN_POINT('Ctrl Pts',(-20.0335231377892,17.5397942632356,
-11.5752265173698));
#106035=CARTESIAN_POINT('Ctrl Pts',(-20.0334982514618,17.5397749120179,
-11.5752246124438));
#106036=CARTESIAN_POINT('Ctrl Pts',(-20.0334856960872,17.5397651493828,
-11.5752236513898));
#106037=CARTESIAN_POINT('Ctrl Pts',(-20.0334603558312,17.5397454461138,
-11.5752217117107));
#106038=CARTESIAN_POINT('Ctrl Pts',(-20.0334475709584,17.5397355054951,
-11.5752207330862));
#106039=CARTESIAN_POINT('Ctrl Pts',(-20.0307420610612,17.5376319409334,
-11.5750136380816));
#106040=CARTESIAN_POINT('Ctrl Pts',(-20.0280443381108,17.5355448724492,
-11.5748070551759));
#106041=CARTESIAN_POINT('Ctrl Pts',(-20.0217183146218,17.5306751951837,
-11.5743224423692));
#106042=CARTESIAN_POINT('Ctrl Pts',(-20.0180860470383,17.5278978253271,
-11.5740440482796));
#106043=CARTESIAN_POINT('Ctrl Pts',(-20.0069159694157,17.5194139637821,
-11.5731875677778));
#106044=CARTESIAN_POINT('Ctrl Pts',(-19.9993490269805,17.5137462725279,
-11.5726068716553));
#106045=CARTESIAN_POINT('Ctrl Pts',(-19.8929714721592,17.4351755328555,
-11.5644394761263));
#106046=CARTESIAN_POINT('Ctrl Pts',(-19.7880493079973,17.3709618075451,
-11.5563504883798));
#106047=CARTESIAN_POINT('Ctrl Pts',(-19.5840730471582,17.2693209845488,
-11.5412923247994));
#106048=CARTESIAN_POINT('Ctrl Pts',(-19.4866077199321,17.2295040114444,
-11.5343486951377));
#106049=CARTESIAN_POINT('Ctrl Pts',(-19.3341667211761,17.1801074084072,
-11.5240486173121));
#106050=CARTESIAN_POINT('Ctrl Pts',(-19.2811053798119,17.1651746564991,
-11.5205596053547));
#106051=CARTESIAN_POINT('Ctrl Pts',(-19.1941608463262,17.1443317532563,
-11.5150022114063));
#106052=CARTESIAN_POINT('Ctrl Pts',(-19.1606128272286,17.1371467364979,
-11.5128953937016));
#106053=CARTESIAN_POINT('Ctrl Pts',(-19.1162828425483,17.1287738719271,
-11.5101589172838));
#106054=CARTESIAN_POINT('Ctrl Pts',(-19.1056469286479,17.1268492407342,
-11.5095059183646));
#106055=CARTESIAN_POINT('Ctrl Pts',(-19.0881996248776,17.1238298564816,
-11.5084404254008));
#106056=CARTESIAN_POINT('Ctrl Pts',(-19.0813968951305,17.1226868095844,
-11.5080264019505));
#106057=CARTESIAN_POINT('Ctrl Pts',(-19.0682159988403,17.1205382434269,
-11.5072268874871));
#106058=CARTESIAN_POINT('Ctrl Pts',(-19.0618385882497,17.1195286157694,
-11.5068412701392));
#106059=CARTESIAN_POINT('Ctrl Pts',(-19.047099958625,17.1172643677929,-11.5059528464782));
#106060=CARTESIAN_POINT('Ctrl Pts',(-19.0387356075384,17.116030622103,-11.505450706246));
#106061=CARTESIAN_POINT('Ctrl Pts',(-19.0162147777684,17.1128465209799,
-11.5041040841106));
#106062=CARTESIAN_POINT('Ctrl Pts',(-19.0020454172619,17.1109893163341,
-11.5032625436985));
#106063=CARTESIAN_POINT('Ctrl Pts',(-18.8718534913555,17.09526400384,-11.4955800345721));
#106064=CARTESIAN_POINT('Ctrl Pts',(-18.7548809745676,17.0908793336759,
-11.4890558161052));
#106065=CARTESIAN_POINT('Ctrl Pts',(-18.4754784123043,17.1035452086983,
-11.4737444116413));
#106066=CARTESIAN_POINT('Ctrl Pts',(-18.3142400771303,17.1296569650721,
-11.4651405278943));
#106067=CARTESIAN_POINT('Ctrl Pts',(-18.1264120002332,17.1828045289622,
-11.4539312087114));
#106068=CARTESIAN_POINT('Ctrl Pts',(-18.0954257233085,17.1923463199269,
-11.4520402013928));
#106069=CARTESIAN_POINT('Ctrl Pts',(-18.0578102079587,17.2048821845487,
-11.4496794072417));
#106070=CARTESIAN_POINT('Ctrl Pts',(-18.0509595891235,17.2072043222906,
-11.449246778347));
#106071=CARTESIAN_POINT('Ctrl Pts',(-18.0402370168989,17.2109003019963,
-11.4485652284902));
#106072=CARTESIAN_POINT('Ctrl Pts',(-18.0363568587799,17.2122504094998,
-11.4483176903531));
#106073=CARTESIAN_POINT('Ctrl Pts',(-18.0291103843932,17.21479550397,-11.4478536548803));
#106074=CARTESIAN_POINT('Ctrl Pts',(-18.0257431542934,17.2159877193328,
-11.4476373224178));
#106075=CARTESIAN_POINT('Ctrl Pts',(-18.0180621558906,17.2187291820401,
-11.4471422359591));
#106076=CARTESIAN_POINT('Ctrl Pts',(-18.0137504064273,17.2202839150778,
-11.4468631593991));
#106077=CARTESIAN_POINT('Ctrl Pts',(-18.0005076293773,17.2251076584017,
-11.446002534179));
#106078=CARTESIAN_POINT('Ctrl Pts',(-17.9915936980599,17.228422807237,-11.445418339707));
#106079=CARTESIAN_POINT('Ctrl Pts',(-17.9106479665844,17.2591494902491,
-11.4400706938159));
#106080=CARTESIAN_POINT('Ctrl Pts',(-17.8401483310086,17.2904127108057,
-11.4351061750814));
#106081=CARTESIAN_POINT('Ctrl Pts',(-17.6517735869652,17.3865686132769,
-11.4212671672486));
#106082=CARTESIAN_POINT('Ctrl Pts',(-17.5381140560914,17.4589656360344,
-11.4122838432954));
#106083=CARTESIAN_POINT('Ctrl Pts',(-17.3615866073959,17.5966380928363,
-11.3977800034907));
#106084=CARTESIAN_POINT('Ctrl Pts',(-17.2946313903948,17.6560387676602,
-11.3921155164201));
#106085=CARTESIAN_POINT('Ctrl Pts',(-17.2170661150255,17.7341697178937,
-11.3853579009784));
#106086=CARTESIAN_POINT('Ctrl Pts',(-17.2027212171555,17.7490487592684,
-11.3840988333214));
#106087=CARTESIAN_POINT('Ctrl Pts',(-17.1825230597481,17.770622527984,-11.3823119452264));
#106088=CARTESIAN_POINT('Ctrl Pts',(-17.1764908649224,17.7771474078774,
-11.3817764395737));
#106089=CARTESIAN_POINT('Ctrl Pts',(-17.1661147309155,17.7885137656125,
-11.3808520030361));
#106090=CARTESIAN_POINT('Ctrl Pts',(-17.1617517269921,17.7933376024162,
-11.3804622639691));
#106091=CARTESIAN_POINT('Ctrl Pts',(-17.1534123993448,17.8026436049007,
-11.3797153062182));
#106092=CARTESIAN_POINT('Ctrl Pts',(-17.1494327430641,17.8071226875738,
-11.3793579491379));
#106093=CARTESIAN_POINT('Ctrl Pts',(-17.1390723605854,17.8188834247486,
-11.3784252275528));
#106094=CARTESIAN_POINT('Ctrl Pts',(-17.1327224291063,17.8261921145004,
-11.3778511501465));
#106095=CARTESIAN_POINT('Ctrl Pts',(-17.1109326916153,17.8516221034012,
-11.3758725496567));
#106096=CARTESIAN_POINT('Ctrl Pts',(-17.0957482120688,17.8699605150712,
-11.3744785031832));
#106097=CARTESIAN_POINT('Ctrl Pts',(-16.9809519754435,18.0134613512361,
-11.3638086918584));
#106098=CARTESIAN_POINT('Ctrl Pts',(-16.8955049454504,18.1492942495825,
-11.355139250804));
#106099=CARTESIAN_POINT('Ctrl Pts',(-16.7687398322938,18.4128784968633,
-11.3392522400741));
#106100=CARTESIAN_POINT('Ctrl Pts',(-16.722658037229,18.5373987086006,-11.3320561440501));
#106101=CARTESIAN_POINT('Ctrl Pts',(-16.6854511075074,18.6768856932822,
-11.3235369086322));
#106102=CARTESIAN_POINT('Ctrl Pts',(-16.6824807208633,18.688410973857,-11.3228296072729));
#106103=CARTESIAN_POINT('Ctrl Pts',(-16.6783955606457,18.7048334219099,
-11.3218161639325));
#106104=CARTESIAN_POINT('Ctrl Pts',(-16.6772007270811,18.7097106966971,
-11.3215144828439));
#106105=CARTESIAN_POINT('Ctrl Pts',(-16.6751713061913,18.7181241428242,
-11.3209927954166));
#106106=CARTESIAN_POINT('Ctrl Pts',(-16.6743284401425,18.7216583336757,
-11.3207732643332));
#106107=CARTESIAN_POINT('Ctrl Pts',(-16.6727116556253,18.7285157988948,
-11.3203465234846));
#106108=CARTESIAN_POINT('Ctrl Pts',(-16.6719366718143,18.7318387816814,
-11.3201393821978));
#106109=CARTESIAN_POINT('Ctrl Pts',(-16.6698670219458,18.7408110594636,
-11.3195791655846));
#106110=CARTESIAN_POINT('Ctrl Pts',(-16.6685875272649,18.7464637726204,
-11.3192252337057));
#106111=CARTESIAN_POINT('Ctrl Pts',(-16.6639224608173,18.7674740157194,
-11.3179062564002));
#106112=CARTESIAN_POINT('Ctrl Pts',(-16.6606849336319,18.782863434113,-11.3169332733319));
#106113=CARTESIAN_POINT('Ctrl Pts',(-16.6315545776624,18.9294197676727,
-11.3076114803182));
#106114=CARTESIAN_POINT('Ctrl Pts',(-16.6179731617444,19.0627150742554,
-11.2987286172781));
#106115=CARTESIAN_POINT('Ctrl Pts',(-16.6159381294442,19.3575225289747,
-11.279257179858));
#106116=CARTESIAN_POINT('Ctrl Pts',(-16.6332267342542,19.5182877290594,
-11.2687827793791));
#106117=CARTESIAN_POINT('Ctrl Pts',(-16.6726949506265,19.6937614786819,
-11.2577663860324));
#106118=CARTESIAN_POINT('Ctrl Pts',(-16.6770300595005,19.7119110207862,
-11.2566312272291));
#106119=CARTESIAN_POINT('Ctrl Pts',(-16.6836951122388,19.738268029812,-11.2549885646297));
#106120=CARTESIAN_POINT('Ctrl Pts',(-16.6858355071368,19.7465221018191,
-11.2544749779631));
#106121=CARTESIAN_POINT('Ctrl Pts',(-16.6896811727935,19.7609918824613,
-11.2535760407691));
#106122=CARTESIAN_POINT('Ctrl Pts',(-16.6913650566072,19.7672131133834,
-11.253190003525));
#106123=CARTESIAN_POINT('Ctrl Pts',(-16.694694150111,19.7792936626221,-11.25244124102));
#106124=CARTESIAN_POINT('Ctrl Pts',(-16.6963362652449,19.7851537613059,
-11.2520784196587));
#106125=CARTESIAN_POINT('Ctrl Pts',(-16.7003292378898,19.7991702841125,
-11.2512115022822));
#106126=CARTESIAN_POINT('Ctrl Pts',(-16.702703938274,19.807319850902,-11.2507081862378));
#106127=CARTESIAN_POINT('Ctrl Pts',(-16.7114937949828,19.836823283509,-11.2488885306869));
#106128=CARTESIAN_POINT('Ctrl Pts',(-16.7181973228101,19.8580902207719,
-11.2475816003458));
#106129=CARTESIAN_POINT('Ctrl Pts',(-16.7832110064602,20.0535224277731,
-11.2356051056296));
#106130=CARTESIAN_POINT('Ctrl Pts',(-16.863615029258,20.2195077983969,-11.2257712892612));
#106131=CARTESIAN_POINT('Ctrl Pts',(-17.0091283207147,20.4410954386816,
-11.2113256851837));
#106132=CARTESIAN_POINT('Ctrl Pts',(-17.0577018893979,20.5065074936038,
-11.2068523316914));
#106133=CARTESIAN_POINT('Ctrl Pts',(-17.1332465148671,20.5968571775584,
-11.200118114807));
#106134=CARTESIAN_POINT('Ctrl Pts',(-17.1572902942947,20.6241517904327,
-11.1980031086553));
#106135=CARTESIAN_POINT('Ctrl Pts',(-17.1871153249824,20.6563002642737,
-11.1953935088133));
#106136=CARTESIAN_POINT('Ctrl Pts',(-17.1922362116198,20.661761685721,-11.1949459226384));
#106137=CARTESIAN_POINT('Ctrl Pts',(-17.2002499741399,20.6702180081735,
-11.1942460064957));
#106138=CARTESIAN_POINT('Ctrl Pts',(-17.2031229576615,20.6732317934441,
-11.193995184822));
#106139=CARTESIAN_POINT('Ctrl Pts',(-17.2084725451051,20.6788105112329,
-11.1935282921086));
#106140=CARTESIAN_POINT('Ctrl Pts',(-17.2109467443891,20.6813776700208,
-11.1933124062761));
#106141=CARTESIAN_POINT('Ctrl Pts',(-17.2165615029321,20.6871740067452,
-11.192822617295));
#106142=CARTESIAN_POINT('Ctrl Pts',(-17.2197058742373,20.6903994019153,
-11.1925484186943));
#106143=CARTESIAN_POINT('Ctrl Pts',(-17.2278442018562,20.6986943071637,
-11.1918390299488));
#106144=CARTESIAN_POINT('Ctrl Pts',(-17.2328534221425,20.7037486688498,
-11.1914026814653));
#106145=CARTESIAN_POINT('Ctrl Pts',(-17.2636240960976,20.7344851254862,
-11.1887245785999));
#106146=CARTESIAN_POINT('Ctrl Pts',(-17.2900168422225,20.7595233291875,
-11.1864373663102));
#106147=CARTESIAN_POINT('Ctrl Pts',(-17.3284016498339,20.7941033287077,
-11.183141132263));
#106148=CARTESIAN_POINT('Ctrl Pts',(-17.3398741119615,20.8042155719893,
-11.1821596154963));
#106149=CARTESIAN_POINT('Ctrl Pts',(-17.3623619963444,20.8236083293833,
-11.1802443075245));
#106150=CARTESIAN_POINT('Ctrl Pts',(-17.3733646504341,20.8329025458702,
-11.1793111067676));
#106151=CARTESIAN_POINT('Ctrl Pts',(-17.5037665382605,20.9407954958032,
-11.1683040397763));
#106152=CARTESIAN_POINT('Ctrl Pts',(-17.6335443859336,21.0261226182628,
-11.15791299429));
#106153=CARTESIAN_POINT('Ctrl Pts',(-17.8260805709793,21.1244078526214,
-11.1439515806298));
#106154=CARTESIAN_POINT('Ctrl Pts',(-17.8818712216058,21.1498978700305,
-11.1400533877699));
#106155=CARTESIAN_POINT('Ctrl Pts',(-17.9730226558238,21.1868478140952,
-11.1339258497592));
#106156=CARTESIAN_POINT('Ctrl Pts',(-18.0077121643375,21.1998608182901,
-11.1316475071957));
#106157=CARTESIAN_POINT('Ctrl Pts',(-18.0532298482721,21.2155858608301,
-11.1287250877809));
#106158=CARTESIAN_POINT('Ctrl Pts',(-18.0637611517557,21.2191315610793,
-11.1280535217017));
#106159=CARTESIAN_POINT('Ctrl Pts',(-18.080938105988,21.2247645521812,-11.1269654885831));
#106160=CARTESIAN_POINT('Ctrl Pts',(-18.0875668985806,21.2269022189148,
-11.1265473654658));
#106161=CARTESIAN_POINT('Ctrl Pts',(-18.1003377952121,21.2309511345486,
-11.1257451589221));
#106162=CARTESIAN_POINT('Ctrl Pts',(-18.1064782878332,21.2328671761296,
-11.12536092163));
#106163=CARTESIAN_POINT('Ctrl Pts',(-18.1205619511819,21.237191415267,-11.124482983632));
#106164=CARTESIAN_POINT('Ctrl Pts',(-18.1285107748232,21.2395809553057,
-11.1239898984634));
#106165=CARTESIAN_POINT('Ctrl Pts',(-18.1496741058157,21.2458075064624,
-11.1226833900505));
#106166=CARTESIAN_POINT('Ctrl Pts',(-18.1629124549513,21.2495625740202,
-11.1218726373307));
#106167=CARTESIAN_POINT('Ctrl Pts',(-18.2646755391493,21.2773586389636,
-11.1156882871355));
#106168=CARTESIAN_POINT('Ctrl Pts',(-18.3546475436367,21.2957537435224,
-11.1105035040751));
#106169=CARTESIAN_POINT('Ctrl Pts',(-18.5850410149184,21.3274426100362,
-11.0976385322787));
#106170=CARTESIAN_POINT('Ctrl Pts',(-18.7261028645048,21.3326629126159,
-11.0901532712794));
#106171=CARTESIAN_POINT('Ctrl Pts',(-18.9197796953218,21.3205047949299,
-11.0794171883434));
#106172=CARTESIAN_POINT('Ctrl Pts',(-18.9727768894575,21.3151647740702,
-11.0764282988209));
#106173=CARTESIAN_POINT('Ctrl Pts',(-19.0530270227582,21.3040079881616,
-11.0717509325949));
#106174=CARTESIAN_POINT('Ctrl Pts',(-19.0804620802739,21.299641792904,-11.0701245936126));
#106175=CARTESIAN_POINT('Ctrl Pts',(-19.1145806000935,21.2935212695761,
-11.068059056357));
#106176=CARTESIAN_POINT('Ctrl Pts',(-19.1213533549372,21.2922721606862,
-11.0676469070562));
#106177=CARTESIAN_POINT('Ctrl Pts',(-19.132081071184,21.2902394561277,-11.0669905363685));
#106178=CARTESIAN_POINT('Ctrl Pts',(-19.1360401643707,21.2894775583973,
-11.0667475336628));
#106179=CARTESIAN_POINT('Ctrl Pts',(-19.1435166158106,21.2880166108967,
-11.0662871495129));
#106180=CARTESIAN_POINT('Ctrl Pts',(-19.1470343830802,21.2873199315696,
-11.0660699038531));
#106181=CARTESIAN_POINT('Ctrl Pts',(-19.1550907644023,21.2857031146373,
-11.0655709405759));
#106182=CARTESIAN_POINT('Ctrl Pts',(-19.1596281368579,21.2847770212648,
-11.0652888863698));
#106183=CARTESIAN_POINT('Ctrl Pts',(-19.1717032312351,21.2822711543069,
-11.0645355729004));
#106184=CARTESIAN_POINT('Ctrl Pts',(-19.1792353518084,21.2806651397423,
-11.0640628742583));
#106185=CARTESIAN_POINT('Ctrl Pts',(-19.2329514076814,21.2689048963913,
-11.0606725719468));
#106186=CARTESIAN_POINT('Ctrl Pts',(-19.2787888660389,21.2572476416358,
-11.057678209601));
#106187=CARTESIAN_POINT('Ctrl Pts',(-19.327919673285,21.2429851071738,-11.0543855819364));
#106188=CARTESIAN_POINT('Ctrl Pts',(-19.3316428036375,21.2418931860235,
-11.0541355428846));
#106189=CARTESIAN_POINT('Ctrl Pts',(-19.3401240257215,21.2393804681468,
-11.0535647930362));
#106190=CARTESIAN_POINT('Ctrl Pts',(-19.34488015232,21.2379531560931,-11.0532438880699));
#106191=CARTESIAN_POINT('Ctrl Pts',(-19.3733564021484,21.2292981137232,
-11.0513176746354));
#106192=CARTESIAN_POINT('Ctrl Pts',(-19.396952521248,21.2216709771324,-11.0497013216415));
#106193=CARTESIAN_POINT('Ctrl Pts',(-19.457529509479,21.2009080112977,-11.0455074332608));
#106194=CARTESIAN_POINT('Ctrl Pts',(-19.4942888383445,21.187155261532,-11.042919375839));
#106195=CARTESIAN_POINT('Ctrl Pts',(-19.6319038481043,21.1312611157895,
-11.0331075129289));
#106196=CARTESIAN_POINT('Ctrl Pts',(-19.7298346063784,21.0823500415907,
-11.0258811690573));
#106197=CARTESIAN_POINT('Ctrl Pts',(-19.8707065449846,20.9977880625475,
-11.0153210767918));
#106198=CARTESIAN_POINT('Ctrl Pts',(-19.9167399310098,20.9676560340767,
-11.0118389064452));
#106199=CARTESIAN_POINT('Ctrl Pts',(-19.989459172803,20.9159001970269,-11.0062911348919));
#106200=CARTESIAN_POINT('Ctrl Pts',(-20.0168825279939,20.8953619121748,
-11.0041872637018));
#106201=CARTESIAN_POINT('Ctrl Pts',(-20.0522837146794,20.8674823423999,
-11.0014539967142));
#106202=CARTESIAN_POINT('Ctrl Pts',(-20.060719583527,20.8607335713784,-11.0008013291272));
#106203=CARTESIAN_POINT('Ctrl Pts',(-20.0744558832739,20.8495708989396,
-10.9997362382166));
#106204=CARTESIAN_POINT('Ctrl Pts',(-20.0797869803167,20.8451952059703,
-10.9993222877143));
#106205=CARTESIAN_POINT('Ctrl Pts',(-20.0900678090611,20.8366724125768,
-10.9985228183528));
#106206=CARTESIAN_POINT('Ctrl Pts',(-20.0950201305242,20.8325285694427,
-10.9981371736606));
#106207=CARTESIAN_POINT('Ctrl Pts',(-20.106414970519,20.8229049847666,-10.9972485500964));
#106208=CARTESIAN_POINT('Ctrl Pts',(-20.1128437930544,20.8174091411412,
-10.9967462382674));
#106209=CARTESIAN_POINT('Ctrl Pts',(-20.1300532723777,20.8025177510998,
-10.9953988519906));
#106210=CARTESIAN_POINT('Ctrl Pts',(-20.1407720696844,20.7930511528646,
-10.9945567243212));
#106211=CARTESIAN_POINT('Ctrl Pts',(-20.2387839193093,20.7047055148721,
-10.986826653984));
#106212=CARTESIAN_POINT('Ctrl Pts',(-20.319460569841,20.618782274522,-10.9802601807293));
#106213=CARTESIAN_POINT('Ctrl Pts',(-20.4942609397657,20.3984081969231,
-10.964865660767));
#106214=CARTESIAN_POINT('Ctrl Pts',(-20.5807193123279,20.2588894181197,
-10.9562205640924));
#106215=CARTESIAN_POINT('Ctrl Pts',(-20.6634192031584,20.0827747350609,
-10.9450300389358));
#106216=CARTESIAN_POINT('Ctrl Pts',(-20.6759748549493,20.0544352876828,
-10.9432201481326));
#106217=CARTESIAN_POINT('Ctrl Pts',(-20.6906487518604,20.0192484431265,
-10.9409496676435));
#106218=CARTESIAN_POINT('Ctrl Pts',(-20.6933610171813,20.0126509745681,
-10.9405229627674));
#106219=CARTESIAN_POINT('Ctrl Pts',(-20.6975744486875,20.0022528560292,
-10.9398486931349));
#106220=CARTESIAN_POINT('Ctrl Pts',(-20.6990980704846,19.998461281868,-10.9396024628172));
#106221=CARTESIAN_POINT('Ctrl Pts',(-20.7019342809556,19.9913438027277,
-10.939139518495));
#106222=CARTESIAN_POINT('Ctrl Pts',(-20.7032494244098,19.988018975572,-10.9389229611091));
#106223=CARTESIAN_POINT('Ctrl Pts',(-20.7062437528034,19.9803925544831,
-10.9384255506059));
#106224=CARTESIAN_POINT('Ctrl Pts',(-20.7079172856637,19.9760887999387,
-10.9381443632281));
#106225=CARTESIAN_POINT('Ctrl Pts',(-20.7130574322784,19.9627409745949,
-10.9372708464959));
#106226=CARTESIAN_POINT('Ctrl Pts',(-20.7164760114298,19.9536787118702,
-10.9366757574526));
#106227=CARTESIAN_POINT('Ctrl Pts',(-20.7565245175941,19.8452677016758,
-10.9295353227033));
#106228=CARTESIAN_POINT('Ctrl Pts',(-20.7857089216245,19.743340227512,-10.9226145524593));
#106229=CARTESIAN_POINT('Ctrl Pts',(-20.8362075146981,19.4991187304815,
-10.9061648543539));
#106230=CARTESIAN_POINT('Ctrl Pts',(-20.8509047690848,19.3559558994674,
-10.8966462544734));
#106231=CARTESIAN_POINT('Ctrl Pts',(-20.8510404641427,19.1504033897853,
-10.8835936337831));
#106232=CARTESIAN_POINT('Ctrl Pts',(-20.8483582574264,19.0884329461174,
-10.8797325916156));
#106233=CARTESIAN_POINT('Ctrl Pts',(-20.8418780039874,19.0142932904846,
-10.8751998038545));
#106234=CARTESIAN_POINT('Ctrl Pts',(-20.8406878629741,19.001931906853,-10.8744468922717));
#106235=CARTESIAN_POINT('Ctrl Pts',(-20.8385539134922,18.9816409475059,
-10.8732155210563));
#106236=CARTESIAN_POINT('Ctrl Pts',(-20.837673901159,18.9737050989499,-10.8727350656425));
#106237=CARTESIAN_POINT('Ctrl Pts',(-20.8360103028502,18.9594401578817,
-10.8718734213025));
#106238=CARTESIAN_POINT('Ctrl Pts',(-20.8352429787225,18.9531092998899,
-10.8714917248528));
#106239=CARTESIAN_POINT('Ctrl Pts',(-20.8335469912293,18.9396267541141,
-10.8706803091881));
#106240=CARTESIAN_POINT('Ctrl Pts',(-20.8326103654351,18.9324761356255,
-10.8702508463239));
#106241=CARTESIAN_POINT('Ctrl Pts',(-20.8299874442421,18.9132163453064,
-10.8690964080671));
#106242=CARTESIAN_POINT('Ctrl Pts',(-20.82823274486,18.9011166489953,-10.8683735993557));
#106243=CARTESIAN_POINT('Ctrl Pts',(-20.8189028582193,18.8404843987702,
-10.8647630646501));
#106244=CARTESIAN_POINT('Ctrl Pts',(-20.8097446634955,18.7922084255718,
-10.8619258576018));
#106245=CARTESIAN_POINT('Ctrl Pts',(-20.7790242557178,18.6562883324648,
-10.8540037395737));
#106246=CARTESIAN_POINT('Ctrl Pts',(-20.75352795488,18.5696444497169,-10.8490364708034));
#106247=CARTESIAN_POINT('Ctrl Pts',(-20.7225806140666,18.4848897181842,
-10.844119113415));
#106248=CARTESIAN_POINT('Origin',(-18.734,19.211,0.));
#106249=CARTESIAN_POINT('',(-20.7225806138021,18.4848897174598,-10.0464612475213));
#106250=CARTESIAN_POINT('',(-20.7219730443074,18.4851210911025,-10.2662522663146));
#106251=CARTESIAN_POINT('',(-20.7225806137986,18.4848897174502,0.));
#106252=CARTESIAN_POINT('',(-20.853822977789,19.2099225630314,-10.3109437209775));
#106253=CARTESIAN_POINT('Ctrl Pts',(-20.7219730443073,18.4851210911022,
-10.2662522663145));
#106254=CARTESIAN_POINT('Ctrl Pts',(-20.7875398406205,18.6593673202803,
-10.2774434393124));
#106255=CARTESIAN_POINT('Ctrl Pts',(-20.8444161789688,18.9018894991261,
-10.2923405908667));
#106256=CARTESIAN_POINT('Ctrl Pts',(-20.8542040821902,19.1485339254976,
-10.307237742421));
#106257=CARTESIAN_POINT('Ctrl Pts',(-20.853822977789,19.2099225630314,-10.3109437209775));
#106258=CARTESIAN_POINT('Ctrl Pts',(-20.8509997772509,19.210028856431,-10.3093226316228));
#106259=CARTESIAN_POINT('Ctrl Pts',(-20.8510795347034,19.3838924485192,
-10.3205062140852));
#106260=CARTESIAN_POINT('Ctrl Pts',(-20.8297420835379,19.5571145591513,
-10.3322367335455));
#106261=CARTESIAN_POINT('Ctrl Pts',(-20.7726128044767,19.7849965017717,
-10.3474068945114));
#106262=CARTESIAN_POINT('Ctrl Pts',(-20.7552168309962,19.8435328169872,
-10.3512871713045));
#106263=CARTESIAN_POINT('Ctrl Pts',(-20.7232747138574,19.9361472779942,
-10.3573899605202));
#106264=CARTESIAN_POINT('Ctrl Pts',(-20.7103236571686,19.9707351732621,
-10.3596609811954));
#106265=CARTESIAN_POINT('Ctrl Pts',(-20.6923110115516,20.015257531746,-10.3625754978198));
#106266=CARTESIAN_POINT('Ctrl Pts',(-20.6880673552092,20.0255139495368,
-10.3632462992183));
#106267=CARTESIAN_POINT('Ctrl Pts',(-20.6810308933608,20.0421487056393,
-10.3643334037274));
#106268=CARTESIAN_POINT('Ctrl Pts',(-20.6782869804511,20.0485473777868,
-10.364751357626));
#106269=CARTESIAN_POINT('Ctrl Pts',(-20.6729469184083,20.0608324746743,
-10.3655534473118));
#106270=CARTESIAN_POINT('Ctrl Pts',(-20.6703554080878,20.0667208203588,
-10.3659377358523));
#106271=CARTESIAN_POINT('Ctrl Pts',(-20.6643565850482,20.080184356458,-10.3668160794057));
#106272=CARTESIAN_POINT('Ctrl Pts',(-20.6609314373623,20.087751521046,-10.3673095169224));
#106273=CARTESIAN_POINT('Ctrl Pts',(-20.6517054951808,20.1078191216519,
-10.3686175786929));
#106274=CARTESIAN_POINT('Ctrl Pts',(-20.6458269701031,20.1202835382805,
-10.3694295221689));
#106275=CARTESIAN_POINT('Ctrl Pts',(-20.5995496897935,20.2159735242317,
-10.3756607081486));
#106276=CARTESIAN_POINT('Ctrl Pts',(-20.5538539910314,20.2965330155285,
-10.38088770432));
#106277=CARTESIAN_POINT('Ctrl Pts',(-20.4258237932771,20.4913033240151,
-10.3937764819646));
#106278=CARTESIAN_POINT('Ctrl Pts',(-20.3371180113939,20.6007678609914,
-10.4012479119931));
#106279=CARTESIAN_POINT('Ctrl Pts',(-20.2010324356082,20.7381864016567,
-10.4119509113538));
#106280=CARTESIAN_POINT('Ctrl Pts',(-20.1624511839615,20.7743326344711,
-10.4149185414929));
#106281=CARTESIAN_POINT('Ctrl Pts',(-20.1087021231141,20.8210373153859,
-10.4190299095633));
#106282=CARTESIAN_POINT('Ctrl Pts',(-20.0946877849398,20.8328985140195,
-10.420099930273));
#106283=CARTESIAN_POINT('Ctrl Pts',(-20.073758755537,20.850149866293,-10.4216980571669));
#106284=CARTESIAN_POINT('Ctrl Pts',(-20.0669616433089,20.8556820540654,
-10.4222171043653));
#106285=CARTESIAN_POINT('Ctrl Pts',(-20.0546538281695,20.8655730056279,
-10.4231574112431));
#106286=CARTESIAN_POINT('Ctrl Pts',(-20.0491553630238,20.8699468746082,
-10.4235776479075));
#106287=CARTESIAN_POINT('Ctrl Pts',(-20.0404397216919,20.8768093517305,
-10.4242441982853));
#106288=CARTESIAN_POINT('Ctrl Pts',(-20.0372369146868,20.8793162428884,
-10.4244892321355));
#106289=CARTESIAN_POINT('Ctrl Pts',(-20.0340175995839,20.8818211277429,
-10.4247356426605));
#106290=CARTESIAN_POINT('Ctrl Pts',(-20.0340082656108,20.8818283901956,
-10.4247363570957));
#106291=CARTESIAN_POINT('Ctrl Pts',(-20.0339895612393,20.8818429431906,
-10.4247377887563));
#106292=CARTESIAN_POINT('Ctrl Pts',(-20.0339801910055,20.8818502336039,
-10.4247385059689));
#106293=CARTESIAN_POINT('Ctrl Pts',(-20.0339614143614,20.8818648423237,
-10.4247399431651));
#106294=CARTESIAN_POINT('Ctrl Pts',(-20.0339520076384,20.8818721608726,
-10.4247406631727));
#106295=CARTESIAN_POINT('Ctrl Pts',(-20.0339331575991,20.8818868261847,
-10.4247421059906));
#106296=CARTESIAN_POINT('Ctrl Pts',(-20.0339237143765,20.8818941728742,
-10.4247428287939));
#106297=CARTESIAN_POINT('Ctrl Pts',(-20.0339041119862,20.8819094229811,
-10.4247443292022));
#106298=CARTESIAN_POINT('Ctrl Pts',(-20.0338939533132,20.8819173259936,
-10.4247451067697));
#106299=CARTESIAN_POINT('Ctrl Pts',(-20.0338734585654,20.8819332697294,
-10.4247466754856));
#106300=CARTESIAN_POINT('Ctrl Pts',(-20.0338631227878,20.8819413102164,
-10.4247474666113));
#106301=CARTESIAN_POINT('Ctrl Pts',(-20.0338422707524,20.8819575312804,
-10.4247490626796));
#106302=CARTESIAN_POINT('Ctrl Pts',(-20.0338317538745,20.8819657123344,
-10.4247498676696));
#106303=CARTESIAN_POINT('Ctrl Pts',(-20.0338105355873,20.8819822176672,
-10.4247514917767));
#106304=CARTESIAN_POINT('Ctrl Pts',(-20.0337998343062,20.8819905418408,
-10.4247523108839));
#106305=CARTESIAN_POINT('Ctrl Pts',(-20.0337782426903,20.8820073369137,
-10.4247539635717));
#106306=CARTESIAN_POINT('Ctrl Pts',(-20.0337673529512,20.8820158073437,
-10.4247547971066));
#106307=CARTESIAN_POINT('Ctrl Pts',(-20.0337453811954,20.8820328974195,
-10.4247564788967));
#106308=CARTESIAN_POINT('Ctrl Pts',(-20.0337342982742,20.8820415177628,
-10.4247573272212));
#106309=CARTESIAN_POINT('Ctrl Pts',(-20.033711935954,20.8820589109134,-10.4247590389118));
#106310=CARTESIAN_POINT('Ctrl Pts',(-20.0337006564343,20.8820676838083,
-10.4247599022873));
#106311=CARTESIAN_POINT('Ctrl Pts',(-20.0336778958689,20.8820853859696,
-10.4247616444667));
#106312=CARTESIAN_POINT('Ctrl Pts',(-20.0336664154454,20.8820943147455,
-10.424762523223));
#106313=CARTESIAN_POINT('Ctrl Pts',(-20.0336432487705,20.8821123319946,
-10.4247642964935));
#106314=CARTESIAN_POINT('Ctrl Pts',(-20.0336315626091,20.8821214203909,
-10.4247651910008));
#106315=CARTESIAN_POINT('Ctrl Pts',(-20.0336079805509,20.8821397598991,
-10.4247669960724));
#106316=CARTESIAN_POINT('Ctrl Pts',(-20.0335960840755,20.8821490114537,
-10.4247679066811));
#106317=CARTESIAN_POINT('Ctrl Pts',(-20.0335720764689,20.8821676810834,
-10.4247697443324));
#106318=CARTESIAN_POINT('Ctrl Pts',(-20.0335599654901,20.8821770990325,
-10.4247706713633));
#106319=CARTESIAN_POINT('Ctrl Pts',(-20.033535524038,20.8821961051915,-10.4247725422296));
#106320=CARTESIAN_POINT('Ctrl Pts',(-20.0335231934309,20.8822056934977,
-10.4247734860753));
#106321=CARTESIAN_POINT('Ctrl Pts',(-20.03349830783,20.8822250441517,-10.4247753909457));
#106322=CARTESIAN_POINT('Ctrl Pts',(-20.0334857528043,20.8822348065163,
-10.424776351973));
#106323=CARTESIAN_POINT('Ctrl Pts',(-20.0334604130318,20.8822545094107,
-10.424778291615));
#106324=CARTESIAN_POINT('Ctrl Pts',(-20.0334476286159,20.8822644496747,
-10.4247792702046));
#106325=CARTESIAN_POINT('Ctrl Pts',(-20.0307421269511,20.8843680079866,
-10.4249863645778));
#106326=CARTESIAN_POINT('Ctrl Pts',(-20.0280444118049,20.886455070613,-10.4251929468845));
#106327=CARTESIAN_POINT('Ctrl Pts',(-20.0217184109835,20.8913247309189,
-10.425677557951));
#106328=CARTESIAN_POINT('Ctrl Pts',(-20.0180861583096,20.8941020897305,
-10.4259559508954));
#106329=CARTESIAN_POINT('Ctrl Pts',(-20.0069161709817,20.9025858840143,
-10.4268124244656));
#106330=CARTESIAN_POINT('Ctrl Pts',(-19.9993493046154,20.908253519964,-10.4273931147414));
#106331=CARTESIAN_POINT('Ctrl Pts',(-19.892968007856,20.9868270576636,-10.4355607974486));
#106332=CARTESIAN_POINT('Ctrl Pts',(-19.7880415525439,21.0510429530457,
-10.4436501165375));
#106333=CARTESIAN_POINT('Ctrl Pts',(-19.5840560713799,21.1526867069838,
-10.4587089149894));
#106334=CARTESIAN_POINT('Ctrl Pts',(-19.4865858912594,21.1925045339,-10.4656528495737));
#106335=CARTESIAN_POINT('Ctrl Pts',(-19.3341454061733,21.2418987269036,
-10.4759527980815));
#106336=CARTESIAN_POINT('Ctrl Pts',(-19.2810897401927,21.2568293634489,
-10.4794414138498));
#106337=CARTESIAN_POINT('Ctrl Pts',(-19.1941536233652,21.2776698097161,
-10.4849982506522));
#106338=CARTESIAN_POINT('Ctrl Pts',(-19.160608252104,21.2848541595246,-10.4871048977934));
#106339=CARTESIAN_POINT('Ctrl Pts',(-19.1162812482732,21.2932264191434,
-10.4898411884362));
#106340=CARTESIAN_POINT('Ctrl Pts',(-19.105645641529,21.2951509871593,-10.4904941681811));
#106341=CARTESIAN_POINT('Ctrl Pts',(-19.0881987131235,21.2981702980181,
-10.4915596378732));
#106342=CARTESIAN_POINT('Ctrl Pts',(-19.0813960508335,21.2993133306391,
-10.4919736570974));
#106343=CARTESIAN_POINT('Ctrl Pts',(-19.0682151944386,21.3014618852634,
-10.4927731689362));
#106344=CARTESIAN_POINT('Ctrl Pts',(-19.0618377561312,21.3024715147506,
-10.4931587878568));
#106345=CARTESIAN_POINT('Ctrl Pts',(-19.0470989310319,21.3047357865575,
-10.4940472230526));
#106346=CARTESIAN_POINT('Ctrl Pts',(-19.0387344119298,21.3059695524934,
-10.4945493731913));
#106347=CARTESIAN_POINT('Ctrl Pts',(-19.0162128344487,21.3091537443846,
-10.495896039452));
#106348=CARTESIAN_POINT('Ctrl Pts',(-19.0020428929694,21.3110110098388,
-10.4967376137776));
#106349=CARTESIAN_POINT('Ctrl Pts',(-18.8718062099437,21.3267415330394,
-10.5044227567239));
#106350=CARTESIAN_POINT('Ctrl Pts',(-18.7547888765673,21.3311240240564,
-10.5109493149571));
#106351=CARTESIAN_POINT('Ctrl Pts',(-18.4752044442039,21.3184318620377,
-10.5262705031869));
#106352=CARTESIAN_POINT('Ctrl Pts',(-18.3138324572534,21.2922716019514,
-10.5348814326682));
#106353=CARTESIAN_POINT('Ctrl Pts',(-18.1260421499104,21.2390820367457,
-10.5460913458496));
#106354=CARTESIAN_POINT('Ctrl Pts',(-18.0952131956695,21.2295838249247,
-10.5479730782015));
#106355=CARTESIAN_POINT('Ctrl Pts',(-18.0577634108762,21.2171020008226,
-10.5503235524921));
#106356=CARTESIAN_POINT('Ctrl Pts',(-18.0509234635446,21.2147833226423,
-10.5507555186146));
#106357=CARTESIAN_POINT('Ctrl Pts',(-18.0402138753413,21.2110916658093,
-10.5514362541201));
#106358=CARTESIAN_POINT('Ctrl Pts',(-18.0363360622653,21.2097423264981,
-10.5516836461284));
#106359=CARTESIAN_POINT('Ctrl Pts',(-18.029091600221,21.2071978636018,-10.5521475582669));
#106360=CARTESIAN_POINT('Ctrl Pts',(-18.0257240426883,21.2060054963237,
-10.5523639144416));
#106361=CARTESIAN_POINT('Ctrl Pts',(-18.018039211939,21.2032625813299,-10.5528592541087));
#106362=CARTESIAN_POINT('Ctrl Pts',(-18.0137239648623,21.2017065266633,
-10.5531385614447));
#106363=CARTESIAN_POINT('Ctrl Pts',(-18.0004598318507,21.1968747782628,
-10.5540005907713));
#106364=CARTESIAN_POINT('Ctrl Pts',(-17.9915281239089,21.1935527278337,
-10.5545859708601));
#106365=CARTESIAN_POINT('Ctrl Pts',(-17.9095482572567,21.1624295455935,
-10.5600022070352));
#106366=CARTESIAN_POINT('Ctrl Pts',(-17.8380772855782,21.1306660400094,
-10.5650397657947));
#106367=CARTESIAN_POINT('Ctrl Pts',(-17.7326832185344,21.0766571319327,
-10.5727922014047));
#106368=CARTESIAN_POINT('Ctrl Pts',(-17.6973643998133,21.0572660540737,
-10.5754488612951));
#106369=CARTESIAN_POINT('Ctrl Pts',(-17.5683033805438,20.9815363820442,
-10.5853336319267));
#106370=CARTESIAN_POINT('Ctrl Pts',(-17.4784083661181,20.9189639352676,
-10.5925644778513));
#106371=CARTESIAN_POINT('Ctrl Pts',(-17.3511186208319,20.8148580617091,
-10.6031340236403));
#106372=CARTESIAN_POINT('Ctrl Pts',(-17.3098649644141,20.7783422763041,
-10.606621114317));
#106373=CARTESIAN_POINT('Ctrl Pts',(-17.2453100661104,20.7165454227837,
-10.6121758063741));
#106374=CARTESIAN_POINT('Ctrl Pts',(-17.2211193680305,20.6922350079567,
-10.6142817968916));
#106375=CARTESIAN_POINT('Ctrl Pts',(-17.1900944257434,20.6595031463752,
-10.6170173723597));
#106376=CARTESIAN_POINT('Ctrl Pts',(-17.1827201608207,20.6516028788732,
-10.6176702783));
#106377=CARTESIAN_POINT('Ctrl Pts',(-17.1707387261679,20.6385681305599,
-10.6187356584339));
#106378=CARTESIAN_POINT('Ctrl Pts',(-17.1660956511109,20.6334670583672,
-10.6191496614082));
#106379=CARTESIAN_POINT('Ctrl Pts',(-17.1571546290361,20.6235471204119,
-10.6199491631924));
#106380=CARTESIAN_POINT('Ctrl Pts',(-17.1528536400138,20.6187311110586,
-10.6203347881965));
#106381=CARTESIAN_POINT('Ctrl Pts',(-17.1429714138387,20.6075631147828,
-10.6212232678859));
#106382=CARTESIAN_POINT('Ctrl Pts',(-17.1374060401068,20.6011971895926,
-10.6217254562207));
#106383=CARTESIAN_POINT('Ctrl Pts',(-17.122536281731,20.5839814157623,-10.6230722925617));
#106384=CARTESIAN_POINT('Ctrl Pts',(-17.1133032857624,20.5730702840548,
-10.623913997595));
#106385=CARTESIAN_POINT('Ctrl Pts',(-17.0294702174267,20.4719407523271,
-10.6316094095525));
#106386=CARTESIAN_POINT('Ctrl Pts',(-16.9623585410229,20.375768297469,-10.6381450905014));
#106387=CARTESIAN_POINT('Ctrl Pts',(-16.8213881891425,20.1331408326455,
-10.653505649878));
#106388=CARTESIAN_POINT('Ctrl Pts',(-16.7559079457202,19.9827300584193,
-10.6621451756692));
#106389=CARTESIAN_POINT('Ctrl Pts',(-16.6992067310605,19.7960675561764,
-10.6733578986754));
#106390=CARTESIAN_POINT('Ctrl Pts',(-16.6907003679106,19.7656296645746,
-10.6752023921982));
#106391=CARTESIAN_POINT('Ctrl Pts',(-16.6811025206306,19.7280613539657,
-10.6775114153712));
#106392=CARTESIAN_POINT('Ctrl Pts',(-16.6793614997114,19.7210991416788,
-10.6779406829497));
#106393=CARTESIAN_POINT('Ctrl Pts',(-16.676682518661,19.7101498341389,-10.6786181023438));
#106394=CARTESIAN_POINT('Ctrl Pts',(-16.6757206536851,19.7061685650602,
-10.6788648988796));
#106395=CARTESIAN_POINT('Ctrl Pts',(-16.673941116773,19.6987080799527,-10.6793283120801));
#106396=CARTESIAN_POINT('Ctrl Pts',(-16.6731206996699,19.6952295761467,
-10.6795447685404));
#106397=CARTESIAN_POINT('Ctrl Pts',(-16.6712638688833,19.6872665622819,
-10.680041156689));
#106398=CARTESIAN_POINT('Ctrl Pts',(-16.6702332725829,19.6827807529395,
-10.6803214175055));
#106399=CARTESIAN_POINT('Ctrl Pts',(-16.6670963897893,19.6689200708493,
-10.6811892618614));
#106400=CARTESIAN_POINT('Ctrl Pts',(-16.665039328775,19.6595343444159,-10.681779554686));
#106401=CARTESIAN_POINT('Ctrl Pts',(-16.6454505617271,19.5671540590612,
-10.6876132465499));
#106402=CARTESIAN_POINT('Ctrl Pts',(-16.6328601615305,19.4831994431482,
-10.6930995615428));
#106403=CARTESIAN_POINT('Ctrl Pts',(-16.6128800721526,19.2587712569526,
-10.7078847396533));
#106404=CARTESIAN_POINT('Ctrl Pts',(-16.6143840936352,19.1179080203136,
-10.7172628525592));
#106405=CARTESIAN_POINT('Ctrl Pts',(-16.6383730535925,18.9010557252902,
-10.7313035421089));
#106406=CARTESIAN_POINT('Ctrl Pts',(-16.6511502936989,18.8244030254141,
-10.7361948925371));
#106407=CARTESIAN_POINT('Ctrl Pts',(-16.6722967670111,18.7299222408223,
-10.7421282458664));
#106408=CARTESIAN_POINT('Ctrl Pts',(-16.676734845176,18.7112839287012,-10.7432941974425));
#106409=CARTESIAN_POINT('Ctrl Pts',(-16.6835354278751,18.6843518106475,
-10.7449728587424));
#106410=CARTESIAN_POINT('Ctrl Pts',(-16.6856964500663,18.6760085536682,
-10.7454920330164));
#106411=CARTESIAN_POINT('Ctrl Pts',(-16.6895661344616,18.6614357258711,
-10.7463974226501));
#106412=CARTESIAN_POINT('Ctrl Pts',(-16.6912524588262,18.6552003900487,
-10.7467843554042));
#106413=CARTESIAN_POINT('Ctrl Pts',(-16.6945759071338,18.6431311043774,
-10.7475324564266));
#106414=CARTESIAN_POINT('Ctrl Pts',(-16.6962095898083,18.6372962798761,
-10.7478937320647));
#106415=CARTESIAN_POINT('Ctrl Pts',(-16.7001643481948,18.6234015927053,
-10.748753162296));
#106416=CARTESIAN_POINT('Ctrl Pts',(-16.7025083271118,18.6153483124574,
-10.7492505675291));
#106417=CARTESIAN_POINT('Ctrl Pts',(-16.7110762478855,18.5865501865974,
-10.7510268739553));
#106418=CARTESIAN_POINT('Ctrl Pts',(-16.717570724429,18.5658867509804,-10.7522969489057));
#106419=CARTESIAN_POINT('Ctrl Pts',(-16.7840604168619,18.3651594669723,
-10.7646007442742));
#106420=CARTESIAN_POINT('Ctrl Pts',(-16.8676918564502,18.1938421500789,
-10.774730972425));
#106421=CARTESIAN_POINT('Ctrl Pts',(-17.0160143725509,17.9715616423399,
-10.7893122345329));
#106422=CARTESIAN_POINT('Ctrl Pts',(-17.0624802662086,17.9095769409566,
-10.7935774807497));
#106423=CARTESIAN_POINT('Ctrl Pts',(-17.1349116915486,17.8232497857898,
-10.8000284415128));
#106424=CARTESIAN_POINT('Ctrl Pts',(-17.1582626137448,17.7967915867878,
-10.8020820436337));
#106425=CARTESIAN_POINT('Ctrl Pts',(-17.1873099291548,17.7654918230145,
-10.8046235111111));
#106426=CARTESIAN_POINT('Ctrl Pts',(-17.1923861853274,17.7600792896601,
-10.805067188069));
#106427=CARTESIAN_POINT('Ctrl Pts',(-17.2003450934466,17.7516820617921,
-10.8057623063219));
#106428=CARTESIAN_POINT('Ctrl Pts',(-17.2032082997816,17.7486789042641,
-10.8060122725733));
#106429=CARTESIAN_POINT('Ctrl Pts',(-17.2085492138833,17.7431098057744,
-10.8064784057865));
#106430=CARTESIAN_POINT('Ctrl Pts',(-17.211024584124,17.7405417023292,-10.8066943927894));
#106431=CARTESIAN_POINT('Ctrl Pts',(-17.2166544045894,17.7347304403955,
-10.8071854928628));
#106432=CARTESIAN_POINT('Ctrl Pts',(-17.2198127531469,17.7314911459828,
-10.8074609081608));
#106433=CARTESIAN_POINT('Ctrl Pts',(-17.2280108528771,17.7231366819758,
-10.8081754993753));
#106434=CARTESIAN_POINT('Ctrl Pts',(-17.2330662422571,17.7180370346621,
-10.8086158615613));
#106435=CARTESIAN_POINT('Ctrl Pts',(-17.2646308497667,17.6865184476744,
-10.8113629830092));
#106436=CARTESIAN_POINT('Ctrl Pts',(-17.2918091070731,17.660782358504,-10.8137178686075));
#106437=CARTESIAN_POINT('Ctrl Pts',(-17.3347064814091,17.6222659328121,
-10.8173994796434));
#106438=CARTESIAN_POINT('Ctrl Pts',(-17.34995242055,17.6089667484124,-10.818701426894));
#106439=CARTESIAN_POINT('Ctrl Pts',(-17.4908527415713,17.4895705784112,
-10.8306580504794));
#106440=CARTESIAN_POINT('Ctrl Pts',(-17.6282823331921,17.3982315275648,
-10.8417216792679));
#106441=CARTESIAN_POINT('Ctrl Pts',(-17.8288125085212,17.2963249868643,
-10.8562402978281));
#106442=CARTESIAN_POINT('Ctrl Pts',(-17.883867081296,17.2712526234096,-10.8600828493431));
#106443=CARTESIAN_POINT('Ctrl Pts',(-17.9739239914241,17.2348120659962,
-10.8661334627554));
#106444=CARTESIAN_POINT('Ctrl Pts',(-18.0082775023838,17.2219395660662,
-10.8683890108845));
#106445=CARTESIAN_POINT('Ctrl Pts',(-18.0534161745131,17.2063510872536,
-10.8712868175459));
#106446=CARTESIAN_POINT('Ctrl Pts',(-18.063910773973,17.202818722488,-10.8719559951208));
#106447=CARTESIAN_POINT('Ctrl Pts',(-18.081042755503,17.197201542884,-10.8730411277717));
#106448=CARTESIAN_POINT('Ctrl Pts',(-18.0876634498147,17.1950668526175,
-10.873458722423));
#106449=CARTESIAN_POINT('Ctrl Pts',(-18.1004290327026,17.1910202372432,
-10.8742605655831));
#106450=CARTESIAN_POINT('Ctrl Pts',(-18.1065723439577,17.1891036252087,
-10.8746449644778));
#106451=CARTESIAN_POINT('Ctrl Pts',(-18.1206770056599,17.1847736776067,
-10.8755241764001));
#106452=CARTESIAN_POINT('Ctrl Pts',(-18.1286440655654,17.1823791875746,
-10.8760183677387));
#106453=CARTESIAN_POINT('Ctrl Pts',(-18.1498877211188,17.1761307266099,
-10.8773297547881));
#106454=CARTESIAN_POINT('Ctrl Pts',(-18.1631884413225,17.1723596952557,
-10.8781442477075));
#106455=CARTESIAN_POINT('Ctrl Pts',(-18.267370450886,17.1439214784324,-10.8844747697419));
#106456=CARTESIAN_POINT('Ctrl Pts',(-18.3597747944633,17.1252110771481,
-10.889791163526));
#106457=CARTESIAN_POINT('Ctrl Pts',(-18.5915301539621,17.0941887716848,
-10.9027105473566));
#106458=CARTESIAN_POINT('Ctrl Pts',(-18.7314188597847,17.0894019203521,
-10.91013447599));
#106459=CARTESIAN_POINT('Ctrl Pts',(-18.9229156420533,17.1017982659259,
-10.9207593955267));
#106460=CARTESIAN_POINT('Ctrl Pts',(-18.9749293575128,17.1071051883609,
-10.9236957143393));
#106461=CARTESIAN_POINT('Ctrl Pts',(-19.0538614279364,17.1181239019138,
-10.9282984953181));
#106462=CARTESIAN_POINT('Ctrl Pts',(-19.0809554862358,17.1224446562798,
-10.9299051564242));
#106463=CARTESIAN_POINT('Ctrl Pts',(-19.1147074886045,17.128502016166,-10.9319486657742));
#106464=CARTESIAN_POINT('Ctrl Pts',(-19.1214525000138,17.1297463869473,
-10.9323591511823));
#106465=CARTESIAN_POINT('Ctrl Pts',(-19.132146355281,17.1317730560228,-10.9330134750114));
#106466=CARTESIAN_POINT('Ctrl Pts',(-19.1360992870879,17.1325338907055,
-10.933256107702));
#106467=CARTESIAN_POINT('Ctrl Pts',(-19.1435709721854,17.1339941045857,
-10.933716211663));
#106468=CARTESIAN_POINT('Ctrl Pts',(-19.1470901266373,17.1346911555874,
-10.9339335495849));
#106469=CARTESIAN_POINT('Ctrl Pts',(-19.1551585924222,17.136310628741,-10.9344332767563));
#106470=CARTESIAN_POINT('Ctrl Pts',(-19.1597066499969,17.1372390700979,
-10.9347160062497));
#106471=CARTESIAN_POINT('Ctrl Pts',(-19.1718288435444,17.1397552552654,
-10.9354722935461));
#106472=CARTESIAN_POINT('Ctrl Pts',(-19.1793973068715,17.1413695683372,
-10.9359473083792));
#106473=CARTESIAN_POINT('Ctrl Pts',(-19.2336956577122,17.1532627493143,
-10.9393747037463));
#106474=CARTESIAN_POINT('Ctrl Pts',(-19.2800703965404,17.1650809667022,
-10.9424056394983));
#106475=CARTESIAN_POINT('Ctrl Pts',(-19.3291631537236,17.1793797921044,
-10.9456979453872));
#106476=CARTESIAN_POINT('Ctrl Pts',(-19.3323233142932,17.1803082311534,
-10.9459102512275));
#106477=CARTESIAN_POINT('Ctrl Pts',(-19.3402000557516,17.1826423602956,
-10.9464403451065));
#106478=CARTESIAN_POINT('Ctrl Pts',(-19.3449139104348,17.1840571257254,
-10.9467584040841));
#106479=CARTESIAN_POINT('Ctrl Pts',(-19.3733511147444,17.1927001714496,
-10.9486819706202));
#106480=CARTESIAN_POINT('Ctrl Pts',(-19.3969503378651,17.200328262934,-10.9502985344721));
#106481=CARTESIAN_POINT('Ctrl Pts',(-19.4575300997938,17.2210922093458,
-10.9544926160063));
#106482=CARTESIAN_POINT('Ctrl Pts',(-19.4942891401823,17.2348448606408,
-10.9570806533823));
#106483=CARTESIAN_POINT('Ctrl Pts',(-19.6319038650052,17.2907388922522,
-10.9668924960268));
#106484=CARTESIAN_POINT('Ctrl Pts',(-19.7298346206829,17.3396499661639,
-10.9741188397263));
#106485=CARTESIAN_POINT('Ctrl Pts',(-19.8707065542806,17.4242119434513,
-10.9846789316369));
#106486=CARTESIAN_POINT('Ctrl Pts',(-19.9167399378574,17.4543439706201,
-10.9881611018028));
#106487=CARTESIAN_POINT('Ctrl Pts',(-19.9894591761601,17.5060998054725,
-10.9937088730945));
#106488=CARTESIAN_POINT('Ctrl Pts',(-20.0168825302285,17.5266380895548,
-10.9958127441997));
#106489=CARTESIAN_POINT('Ctrl Pts',(-20.0522837156195,17.5545176583499,
-10.998546011088));
#106490=CARTESIAN_POINT('Ctrl Pts',(-20.0607195842579,17.5612664292112,
-10.999198678659));
#106491=CARTESIAN_POINT('Ctrl Pts',(-20.0744558836948,17.5724291014053,
-11.0002637695457));
#106492=CARTESIAN_POINT('Ctrl Pts',(-20.0797869806361,17.5768047942932,
-11.0006777200402));
#106493=CARTESIAN_POINT('Ctrl Pts',(-20.0900678092054,17.5853275875439,
-11.0014771893881));
#106494=CARTESIAN_POINT('Ctrl Pts',(-20.0950201305943,17.5894714306165,
-11.0018628340745));
#106495=CARTESIAN_POINT('Ctrl Pts',(-20.1064149704466,17.5990950151723,
-11.0027514576276));
#106496=CARTESIAN_POINT('Ctrl Pts',(-20.1128437929147,17.6045908587393,
-11.0032537694513));
#106497=CARTESIAN_POINT('Ctrl Pts',(-20.1300532721182,17.6194822486732,
-11.0046011557186));
#106498=CARTESIAN_POINT('Ctrl Pts',(-20.1407720693722,17.6289488468585,
-11.0054432833836));
#106499=CARTESIAN_POINT('Ctrl Pts',(-20.2387839238738,17.7172944892056,
-11.0131733541038));
#106500=CARTESIAN_POINT('Ctrl Pts',(-20.3194605785722,17.8032177347584,
-11.0197398277044));
#106501=CARTESIAN_POINT('Ctrl Pts',(-20.4942609474718,18.0235918151934,
-11.0351343477121));
#106502=CARTESIAN_POINT('Ctrl Pts',(-20.5807193165826,18.1631105901631,
-11.043779444138));
#106503=CARTESIAN_POINT('Ctrl Pts',(-20.6634192044316,18.3392252677977,
-11.0549699689516));
#106504=CARTESIAN_POINT('Ctrl Pts',(-20.6759748557222,18.3675647141389,
-11.0567798596891));
#106505=CARTESIAN_POINT('Ctrl Pts',(-20.690648752115,18.4027515574913,-11.0590503401007));
#106506=CARTESIAN_POINT('Ctrl Pts',(-20.6933610173737,18.4093490259035,
-11.0594770449673));
#106507=CARTESIAN_POINT('Ctrl Pts',(-20.6975744487915,18.4197471442292,
-11.0601513145861));
#106508=CARTESIAN_POINT('Ctrl Pts',(-20.6990980705593,18.4235387183188,
-11.0603975448992));
#106509=CARTESIAN_POINT('Ctrl Pts',(-20.70193428098,18.4306561973342,-11.0608604892132));
#106510=CARTESIAN_POINT('Ctrl Pts',(-20.703249424413,18.4339810244365,-11.0610770465957));
#106511=CARTESIAN_POINT('Ctrl Pts',(-20.7062437527631,18.4416074454138,
-11.0615744570916));
#106512=CARTESIAN_POINT('Ctrl Pts',(-20.7079172856,18.4459111998975,-11.0618556444654));
#106513=CARTESIAN_POINT('Ctrl Pts',(-20.7130574321558,18.4592590250836,
-11.0627291611873));
#106514=CARTESIAN_POINT('Ctrl Pts',(-20.7164760112716,18.4683212877087,
-11.0633242502241));
#106515=CARTESIAN_POINT('Ctrl Pts',(-20.7207530739769,18.4798992648316,
-11.06408682766));
#106516=CARTESIAN_POINT('Ctrl Pts',(-20.7216692101372,18.4823936783584,
-11.064251255848));
#106517=CARTESIAN_POINT('Ctrl Pts',(-20.7225806135353,18.4848897167291,
-11.0644159212905));
#106518=CARTESIAN_POINT('',(-20.8509993992227,19.2094051048361,-10.0879365117025));
#106519=CARTESIAN_POINT('Ctrl Pts',(-20.7225806140666,18.4848897181842,
-10.844119113415));
#106520=CARTESIAN_POINT('Ctrl Pts',(-20.7216543340203,18.4823529374921,
-10.8439719327555));
#106521=CARTESIAN_POINT('Ctrl Pts',(-20.7207231706843,18.4798178494646,
-10.8438247920179));
#106522=CARTESIAN_POINT('Ctrl Pts',(-20.6623499375528,18.3218318044859,
-10.8346510877151));
#106523=CARTESIAN_POINT('Ctrl Pts',(-20.5868669459257,18.1736858755523,
-10.8258506394662));
#106524=CARTESIAN_POINT('Ctrl Pts',(-20.4871421987,18.0242494119213,-10.8152892621795));
#106525=CARTESIAN_POINT('Ctrl Pts',(-20.4792655419488,18.0126959100725,
-10.8144606017706));
#106526=CARTESIAN_POINT('Ctrl Pts',(-20.4681194501686,17.9966898135209,
-10.813294299669));
#106527=CARTESIAN_POINT('Ctrl Pts',(-20.4649459698207,17.9921704202635,
-10.8129629302029));
#106528=CARTESIAN_POINT('Ctrl Pts',(-20.4598136886024,17.9849219450265,
-10.812428049678));
#106529=CARTESIAN_POINT('Ctrl Pts',(-20.4578659862623,17.9821849831245,
-10.8122252965722));
#106530=CARTESIAN_POINT('Ctrl Pts',(-20.4537748176495,17.9764648362565,
-10.8117998739036));
#106531=CARTESIAN_POINT('Ctrl Pts',(-20.4516300990772,17.9734825916516,
-10.8115771150017));
#106532=CARTESIAN_POINT('Ctrl Pts',(-20.4464076165922,17.9662604270335,
-10.8110353472665));
#106533=CARTESIAN_POINT('Ctrl Pts',(-20.443321864516,17.9620263365432,-10.81071579051));
#106534=CARTESIAN_POINT('Ctrl Pts',(-20.4323912730453,17.9471443900344,
-10.8095858946531));
#106535=CARTESIAN_POINT('Ctrl Pts',(-20.424462587658,17.9365588916631,-10.8087700182273));
#106536=CARTESIAN_POINT('Ctrl Pts',(-20.3764349043982,17.873674424813,-10.8038532717267));
#106537=CARTESIAN_POINT('Ctrl Pts',(-20.3340141805246,17.8232013633744,
-10.799615538571));
#106538=CARTESIAN_POINT('Ctrl Pts',(-20.2240817870232,17.7041520603046,
-10.7890379008404));
#106539=CARTESIAN_POINT('Ctrl Pts',(-20.1541137676121,17.6380374577248,
-10.7826422294064));
#106540=CARTESIAN_POINT('Ctrl Pts',(-19.9712621264858,17.4874345144272,
-10.7670586891983));
#106541=CARTESIAN_POINT('Ctrl Pts',(-19.8539618981669,17.4090027263477,
-10.7580101507407));
#106542=CARTESIAN_POINT('Ctrl Pts',(-19.7171141043647,17.3360653819244,
-10.7485415016082));
#106543=CARTESIAN_POINT('Ctrl Pts',(-19.7044367172556,17.3294724934841,
-10.7476735710945));
#106544=CARTESIAN_POINT('Ctrl Pts',(-19.684153555759,17.3191837574311,-10.7462993207281));
#106545=CARTESIAN_POINT('Ctrl Pts',(-19.6765908816755,17.3154043394778,
-10.7457900731935));
#106546=CARTESIAN_POINT('Ctrl Pts',(-19.663212876976,17.3088185896121,-10.744894710243));
#106547=CARTESIAN_POINT('Ctrl Pts',(-19.6574070057459,17.3059933879549,
-10.7445079387702));
#106548=CARTESIAN_POINT('Ctrl Pts',(-19.6453717557756,17.3002048494976,
-10.7437098670655));
#106549=CARTESIAN_POINT('Ctrl Pts',(-19.6391406295207,17.29724530649,-10.7432987022512));
#106550=CARTESIAN_POINT('Ctrl Pts',(-19.6231088244508,17.289726637406,-10.7422459640215));
#106551=CARTESIAN_POINT('Ctrl Pts',(-19.6132874162419,17.2852119842185,
-10.7416059320709));
#106552=CARTESIAN_POINT('Ctrl Pts',(-19.5721500222677,17.2666824799479,
-10.7389450419825));
#106553=CARTESIAN_POINT('Ctrl Pts',(-19.5405292253946,17.2533542496531,
-10.7369477176546));
#106554=CARTESIAN_POINT('Ctrl Pts',(-19.45730612924,17.2206345451399,-10.7318030204427));
#106555=CARTESIAN_POINT('Ctrl Pts',(-19.4052449918637,17.2024788507419,
-10.7286950489945));
#106556=CARTESIAN_POINT('Ctrl Pts',(-19.2479504540769,17.15442470414,-10.7195499188603));
#106557=CARTESIAN_POINT('Ctrl Pts',(-19.1410480683381,17.1306250891409,
-10.7136614871618));
#106558=CARTESIAN_POINT('Ctrl Pts',(-18.986908990109,17.1086504772908,-10.705184626503));
#106559=CARTESIAN_POINT('Ctrl Pts',(-18.9408309213161,17.103618403317,-10.7026506559916));
#106560=CARTESIAN_POINT('Ctrl Pts',(-18.8732954417683,17.0984793676563,
-10.6988935198717));
#106561=CARTESIAN_POINT('Ctrl Pts',(-18.8519416472176,17.0971796748016,
-10.6976992482264));
#106562=CARTESIAN_POINT('Ctrl Pts',(-18.7787716411238,17.0938383603343,
-10.6935748127765));
#106563=CARTESIAN_POINT('Ctrl Pts',(-18.7269059588419,17.0933771253771,
-10.6905961530558));
#106564=CARTESIAN_POINT('Ctrl Pts',(-18.6664285235738,17.0950609626963,
-10.6870053840491));
#106565=CARTESIAN_POINT('Ctrl Pts',(-18.6577783141055,17.0953549062234,
-10.6864889766077));
#106566=CARTESIAN_POINT('Ctrl Pts',(-18.6446646876146,17.0958810492267,
-10.6857015161395));
#106567=CARTESIAN_POINT('Ctrl Pts',(-18.6401996825508,17.0960743574386,
-10.6854325892211));
#106568=CARTESIAN_POINT('Ctrl Pts',(-18.6321761206969,17.0964471883601,
-10.6849478255204));
#106569=CARTESIAN_POINT('Ctrl Pts',(-18.6286173788257,17.0966215574175,
-10.6847322800897));
#106570=CARTESIAN_POINT('Ctrl Pts',(-18.6208738567738,17.0970205681956,
-10.6842620957299));
#106571=CARTESIAN_POINT('Ctrl Pts',(-18.6166893520786,17.0972486490708,
-10.6840072715993));
#106572=CARTESIAN_POINT('Ctrl Pts',(-18.6049073397474,17.0979259337829,
-10.6832877436521));
#106573=CARTESIAN_POINT('Ctrl Pts',(-18.5973116276153,17.0984036805232,
-10.6828214861814));
#106574=CARTESIAN_POINT('Ctrl Pts',(-18.5512928651302,17.1015473351933,
-10.6799828602673));
#106575=CARTESIAN_POINT('Ctrl Pts',(-18.5129484348214,17.1052202829683,
-10.677559382916));
#106576=CARTESIAN_POINT('Ctrl Pts',(-18.3856334166693,17.1209309761825,
-10.6693644419136));
#106577=CARTESIAN_POINT('Ctrl Pts',(-18.2973333024692,17.1375805989713,
-10.6634418599992));
#106578=CARTESIAN_POINT('Ctrl Pts',(-18.0441499013831,17.202213570861,-10.6461748034108));
#106579=CARTESIAN_POINT('Ctrl Pts',(-17.8836772629773,17.2646985604323,
-10.6349283640233));
#106580=CARTESIAN_POINT('Ctrl Pts',(-17.7119975759407,17.3568853964835,
-10.6229309391828));
#106581=CARTESIAN_POINT('Ctrl Pts',(-17.6916892526373,17.3682253823639,
-10.6215108978118));
#106582=CARTESIAN_POINT('Ctrl Pts',(-17.6632763130112,17.3847109331125,
-10.619522233943));
#106583=CARTESIAN_POINT('Ctrl Pts',(-17.6550140522053,17.3895801420575,
-10.618943709519));
#106584=CARTESIAN_POINT('Ctrl Pts',(-17.6416583794255,17.3975738277824,
-10.6180080744736));
#106585=CARTESIAN_POINT('Ctrl Pts',(-17.6365446752666,17.4006639788495,
-10.6176497197478));
#106586=CARTESIAN_POINT('Ctrl Pts',(-17.6258801221134,17.4071702363243,
-10.6169021096835));
#106587=CARTESIAN_POINT('Ctrl Pts',(-17.6203318218453,17.4105904158996,
-10.616513008755));
#106588=CARTESIAN_POINT('Ctrl Pts',(-17.6071922927949,17.4187740917833,
-10.6155911255955));
#106589=CARTESIAN_POINT('Ctrl Pts',(-17.5996153035212,17.4235603005258,
-10.6150591880569));
#106590=CARTESIAN_POINT('Ctrl Pts',(-17.5742940552263,17.4397810082951,
-10.6132802211099));
#106591=CARTESIAN_POINT('Ctrl Pts',(-17.5566901147835,17.4514329860545,
-10.6120412883748));
#106592=CARTESIAN_POINT('Ctrl Pts',(-17.4624597246945,17.5158511046683,
-10.6053927119669));
#106593=CARTESIAN_POINT('Ctrl Pts',(-17.3891963448101,17.5733643631854,
-10.6001686665427));
#106594=CARTESIAN_POINT('Ctrl Pts',(-17.2047797618198,17.7388848584874,
-10.5865221978904));
#106595=CARTESIAN_POINT('Ctrl Pts',(-17.1013027708117,17.8545594954077,
-10.5783387053207));
#106596=CARTESIAN_POINT('Ctrl Pts',(-16.9801993074224,18.024093718978,-10.5666244076512));
#106597=CARTESIAN_POINT('Ctrl Pts',(-16.950707137834,18.0688840146192,-10.5635486459546));
#106598=CARTESIAN_POINT('Ctrl Pts',(-16.9184237280195,18.1222171132852,
-10.5598491744357));
#106599=CARTESIAN_POINT('Ctrl Pts',(-16.9139446751054,18.1297211358079,
-10.5593278237063));
#106600=CARTESIAN_POINT('Ctrl Pts',(-16.9072363226249,18.1411198183784,
-10.5585342976682));
#106601=CARTESIAN_POINT('Ctrl Pts',(-16.9049726711123,18.144994293949,-10.5582642978902));
#106602=CARTESIAN_POINT('Ctrl Pts',(-16.900933153481,18.1519590942489,-10.5577783953199));
#106603=CARTESIAN_POINT('Ctrl Pts',(-16.8991527593703,18.1550467306166,
-10.5575627899971));
#106604=CARTESIAN_POINT('Ctrl Pts',(-16.8953029020148,18.1617624544132,
-10.5570934057404));
#106605=CARTESIAN_POINT('Ctrl Pts',(-16.8932364031233,18.1653921265951,
-10.5568394466927));
#106606=CARTESIAN_POINT('Ctrl Pts',(-16.8874664541485,18.1755967884846,
-10.5561247499005));
#106607=CARTESIAN_POINT('Ctrl Pts',(-16.8837874425121,18.1821854226602,
-10.5556624910248));
#106608=CARTESIAN_POINT('Ctrl Pts',(-16.8620940873218,18.2215281189502,
-10.5528980123702));
#106609=CARTESIAN_POINT('Ctrl Pts',(-16.8449158083539,18.2547328461959,
-10.5505476722786));
#106610=CARTESIAN_POINT('Ctrl Pts',(-16.7914642396141,18.365118866017,-10.5427202437643));
#106611=CARTESIAN_POINT('Ctrl Pts',(-16.758974926751,18.4440357485269,-10.5371054176708));
#106612=CARTESIAN_POINT('Ctrl Pts',(-16.6736475831275,18.6930227718753,
-10.5197177477906));
#106613=CARTESIAN_POINT('Ctrl Pts',(-16.6374020638314,18.8679926917734,
-10.508024687605));
#106614=CARTESIAN_POINT('Ctrl Pts',(-16.6216995381932,19.0681871115291,
-10.4956668419621));
#106615=CARTESIAN_POINT('Ctrl Pts',(-16.6202840116311,19.0909435700787,
-10.4942752570022));
#106616=CARTESIAN_POINT('Ctrl Pts',(-16.6187991059411,19.1232235659733,
-10.4923192372809));
#106617=CARTESIAN_POINT('Ctrl Pts',(-16.6184259692592,19.1327309149415,
-10.4917453344423));
#106618=CARTESIAN_POINT('Ctrl Pts',(-16.6179233222142,19.1481985026732,
-10.4908151403365));
#106619=CARTESIAN_POINT('Ctrl Pts',(-16.6177548727037,19.1541572637932,
-10.4904576333428));
#106620=CARTESIAN_POINT('Ctrl Pts',(-16.6174546507248,19.1666443936419,
-10.489710180215));
#106621=CARTESIAN_POINT('Ctrl Pts',(-16.6173279087249,19.1731728292861,
-10.4893203955717));
#106622=CARTESIAN_POINT('Ctrl Pts',(-16.6170979078866,19.1887283122697,
-10.4883939629391));
#106623=CARTESIAN_POINT('Ctrl Pts',(-16.6170221806385,19.1977556863427,
-10.4878581823956));
#106624=CARTESIAN_POINT('Ctrl Pts',(-16.6169613826195,19.2282799081068,
-10.4860526310735));
#106625=CARTESIAN_POINT('Ctrl Pts',(-16.6172459888386,19.249776397744,-10.4847912964629));
#106626=CARTESIAN_POINT('Ctrl Pts',(-16.622968798079,19.4507254041479,-10.4730865891205));
#106627=CARTESIAN_POINT('Ctrl Pts',(-16.6508849994117,19.6288036369092,
-10.4634407893317));
#106628=CARTESIAN_POINT('Ctrl Pts',(-16.7345162291315,19.9168694929822,
-10.4471157906244));
#106629=CARTESIAN_POINT('Ctrl Pts',(-16.7778863883128,20.0294119810515,
-10.440509532291));
#106630=CARTESIAN_POINT('Ctrl Pts',(-16.8347330806377,20.1461814779287,
-10.4328125536686));
#106631=CARTESIAN_POINT('Ctrl Pts',(-16.8389481968708,20.1546937445466,
-10.4322463615213));
#106632=CARTESIAN_POINT('Ctrl Pts',(-16.8452808961623,20.1672688609738,
-10.4314019266966));
#106633=CARTESIAN_POINT('Ctrl Pts',(-16.8473546806142,20.1713538023063,
-10.4311263575692));
#106634=CARTESIAN_POINT('Ctrl Pts',(-16.8510689186138,20.1786116479274,
-10.4306344418552));
#106635=CARTESIAN_POINT('Ctrl Pts',(-16.8527041589658,20.1817871634565,
-10.4304184243771));
#106636=CARTESIAN_POINT('Ctrl Pts',(-16.8562382689555,20.18860767827,-10.429952734729));
#106637=CARTESIAN_POINT('Ctrl Pts',(-16.8581396908201,20.192251237435,-10.4297029070488));
#106638=CARTESIAN_POINT('Ctrl Pts',(-16.8634201712418,20.2022984055287,
-10.4290111384764));
#106639=CARTESIAN_POINT('Ctrl Pts',(-16.8668214536686,20.2086901809639,
-10.4285678265664));
#106640=CARTESIAN_POINT('Ctrl Pts',(-16.8856796893083,20.2436948471861,
-10.4261227917617));
#106641=CARTESIAN_POINT('Ctrl Pts',(-16.9017607057491,20.2719644283098,
-10.4240847631223));
#106642=CARTESIAN_POINT('Ctrl Pts',(-17.0021764420717,20.439394421619,-10.4116790900861));
#106643=CARTESIAN_POINT('Ctrl Pts',(-17.1016737565232,20.5688205528447,
-10.4007212871873));
#106644=CARTESIAN_POINT('Ctrl Pts',(-17.2963388132869,20.7693490770264,
-10.3824661528239));
#106645=CARTESIAN_POINT('Ctrl Pts',(-17.3844667800199,20.8462643261838,
-10.3750285790364));
#106646=CARTESIAN_POINT('Ctrl Pts',(-17.4911520102363,20.9248449959051,
-10.3669377150156));
#106647=CARTESIAN_POINT('Ctrl Pts',(-17.503904462694,20.9340208314554,-10.365983920476));
#106648=CARTESIAN_POINT('Ctrl Pts',(-17.5233533538149,20.947688998477,-10.3645490071438));
#106649=CARTESIAN_POINT('Ctrl Pts',(-17.5299750473181,20.9522862761405,
-10.3640638718326));
#106650=CARTESIAN_POINT('Ctrl Pts',(-17.5418881103604,20.9604567742544,
-10.3631970851697));
#106651=CARTESIAN_POINT('Ctrl Pts',(-17.5471696634533,20.9640440713344,
-10.3628149011501));
#106652=CARTESIAN_POINT('Ctrl Pts',(-17.5584111989841,20.971605373997,-10.362005840726));
#106653=CARTESIAN_POINT('Ctrl Pts',(-17.5643752968711,20.9755731403905,
-10.3615792031245));
#106654=CARTESIAN_POINT('Ctrl Pts',(-17.5803902667297,20.9861106333292,
-10.3604404477912));
#106655=CARTESIAN_POINT('Ctrl Pts',(-17.5904771796444,20.9926253100861,
-10.3597303948442));
#106656=CARTESIAN_POINT('Ctrl Pts',(-17.6398585863886,21.0239263469489,
-10.3562883066337));
#106657=CARTESIAN_POINT('Ctrl Pts',(-17.6799080450982,21.0475015638419,
-10.3536011745934));
#106658=CARTESIAN_POINT('Ctrl Pts',(-17.869069707589,21.1506234581316,-10.3413281212276));
#106659=CARTESIAN_POINT('Ctrl Pts',(-18.0265804656648,21.2134492192743,
-10.3323387424235));
#106660=CARTESIAN_POINT('Ctrl Pts',(-18.2858254415672,21.2823964472521,
-10.3176550200653));
#106661=CARTESIAN_POINT('Ctrl Pts',(-18.3834250818174,21.301128155566,-10.3121334802109));
#106662=CARTESIAN_POINT('Ctrl Pts',(-18.4915899250137,21.3140977985747,
-10.3056794510721));
#106663=CARTESIAN_POINT('Ctrl Pts',(-18.5012236736348,21.3151858683672,
-10.3051017122815));
#106664=CARTESIAN_POINT('Ctrl Pts',(-18.5154581592575,21.3166946131921,
-10.3042433288564));
#106665=CARTESIAN_POINT('Ctrl Pts',(-18.5200535020191,21.3171664785234,
-10.3039654875614));
#106666=CARTESIAN_POINT('Ctrl Pts',(-18.5282085021999,21.3179768971809,
-10.3034710749827));
#106667=CARTESIAN_POINT('Ctrl Pts',(-18.5317675116668,21.3183214767269,
-10.3032548456809));
#106668=CARTESIAN_POINT('Ctrl Pts',(-18.5393945371849,21.3190404175898,
-10.3027904648566));
#106669=CARTESIAN_POINT('Ctrl Pts',(-18.5434627074604,21.3194120156766,
-10.3025421670823));
#106670=CARTESIAN_POINT('Ctrl Pts',(-18.5546322905618,21.3203996858653,
-10.3018588348985));
#106671=CARTESIAN_POINT('Ctrl Pts',(-18.5617357031844,21.3209916631655,
-10.3014224829616));
#106672=CARTESIAN_POINT('Ctrl Pts',(-18.5996701014527,21.3239601697813,
-10.2990832227456));
#106673=CARTESIAN_POINT('Ctrl Pts',(-18.6305456747066,21.3256967087688,
-10.2971475420398));
#106674=CARTESIAN_POINT('Ctrl Pts',(-18.7241033582773,21.3289049998071,
-10.2912081873798));
#106675=CARTESIAN_POINT('Ctrl Pts',(-18.7868208341602,21.3282690883687,
-10.2871270836676));
#106676=CARTESIAN_POINT('Ctrl Pts',(-18.9713807215036,21.3181924241045,
-10.2749807343996));
#106677=CARTESIAN_POINT('Ctrl Pts',(-19.0925523315125,21.3009887310576,
-10.2668443026107));
#106678=CARTESIAN_POINT('Ctrl Pts',(-19.3061139796514,21.2515374903664,
-10.2526438938305));
#106679=CARTESIAN_POINT('Ctrl Pts',(-19.3990545859024,21.2231666539092,
-10.2465102883386));
#106680=CARTESIAN_POINT('Ctrl Pts',(-19.5027250957551,21.1835476434987,
-10.2397370251966));
#106681=CARTESIAN_POINT('Ctrl Pts',(-19.5156692473789,21.1784541115143,
-10.238892417675));
#106682=CARTESIAN_POINT('Ctrl Pts',(-19.5362964385011,21.1701015915325,
-10.237548035836));
#106683=CARTESIAN_POINT('Ctrl Pts',(-19.5440118748617,21.166924177179,-10.2370455285622));
#106684=CARTESIAN_POINT('Ctrl Pts',(-19.5576477703087,21.1612140427079,
-10.2361579762615));
#106685=CARTESIAN_POINT('Ctrl Pts',(-19.5635758012032,21.1586997852309,
-10.2357723112204));
#106686=CARTESIAN_POINT('Ctrl Pts',(-19.5696170997966,21.1561049023048,
-10.2353794495631));
#106687=CARTESIAN_POINT('Ctrl Pts',(-19.5697418750956,21.1560512940934,
-10.2353713355829));
#106688=CARTESIAN_POINT('Ctrl Pts',(-19.5699732862728,21.1559518446766,
-10.2353562873453));
#106689=CARTESIAN_POINT('Ctrl Pts',(-19.5700799230437,21.1559060069206,
-10.2353493530096));
#106690=CARTESIAN_POINT('Ctrl Pts',(-19.5702777089093,21.155820969505,-10.2353364915663));
#106691=CARTESIAN_POINT('Ctrl Pts',(-19.5703688582651,21.155781772531,-10.2353305644271));
#106692=CARTESIAN_POINT('Ctrl Pts',(-19.5705379316014,21.155709051809,-10.2353195702246));
#106693=CARTESIAN_POINT('Ctrl Pts',(-19.5706158554099,21.1556755301778,
-10.2353145031619));
#106694=CARTESIAN_POINT('Ctrl Pts',(-19.5707604075466,21.155613335762,-10.2353051035888));
#106695=CARTESIAN_POINT('Ctrl Pts',(-19.5708270352755,21.1555846647273,
-10.2353007711095));
#106696=CARTESIAN_POINT('Ctrl Pts',(-19.5709506415334,21.1555314673423,
-10.2352927336312));
#106697=CARTESIAN_POINT('Ctrl Pts',(-19.5710076192507,21.1555069424313,
-10.2352890286793));
#106698=CARTESIAN_POINT('Ctrl Pts',(-19.5711339322195,21.1554525669773,
-10.2352808152665));
#106699=CARTESIAN_POINT('Ctrl Pts',(-19.5712032692351,21.1554227142473,
-10.2352763066982));
#106700=CARTESIAN_POINT('Ctrl Pts',(-19.5713395177064,21.1553640444614,
-10.2352674473265));
#106701=CARTESIAN_POINT('Ctrl Pts',(-19.5714064289843,21.1553352277843,
-10.235263096533));
#106702=CARTESIAN_POINT('Ctrl Pts',(-19.5715379181781,21.1552785912924,
-10.2352545467108));
#106703=CARTESIAN_POINT('Ctrl Pts',(-19.5716024959016,21.1552507718407,
-10.2352503476932));
#106704=CARTESIAN_POINT('Ctrl Pts',(-19.571729405952,21.1551960927359,-10.2352420956988));
#106705=CARTESIAN_POINT('Ctrl Pts',(-19.5717917376581,21.1551692336106,
-10.235238042761));
#106706=CARTESIAN_POINT('Ctrl Pts',(-19.5719142399558,21.1551164396126,
-10.235230077442));
#106707=CARTESIAN_POINT('Ctrl Pts',(-19.5719744099628,21.1550905052337,
-10.2352261650975));
#106708=CARTESIAN_POINT('Ctrl Pts',(-19.5720926696469,21.1550395266262,
-10.2352184757084));
#106709=CARTESIAN_POINT('Ctrl Pts',(-19.5721507587247,21.1550144828807,
-10.2352146987017));
#106710=CARTESIAN_POINT('Ctrl Pts',(-19.572264934109,21.154965252769,-10.2352072749419));
#106711=CARTESIAN_POINT('Ctrl Pts',(-19.5723210198019,21.1549410668763,
-10.2352036282276));
#106712=CARTESIAN_POINT('Ctrl Pts',(-19.5724312628441,21.1548935209943,
-10.23519646021));
#106713=CARTESIAN_POINT('Ctrl Pts',(-19.5724854195906,21.1548701614593,
-10.2351929389449));
#106714=CARTESIAN_POINT('Ctrl Pts',(-19.5725918762277,21.154824238034,-10.2351860171745));
#106715=CARTESIAN_POINT('Ctrl Pts',(-19.5726441754442,21.1548016746152,
-10.2351826167121));
#106716=CARTESIAN_POINT('Ctrl Pts',(-19.5727469857355,21.154757314313,-10.2351759320767));
#106717=CARTESIAN_POINT('Ctrl Pts',(-19.572797495968,21.154735517961,-10.2351726479576));
#106718=CARTESIAN_POINT('Ctrl Pts',(-19.5728967944376,21.1546926637473,
-10.2351661917052));
#106719=CARTESIAN_POINT('Ctrl Pts',(-19.5729455814446,21.1546716065727,
-10.2351630196512));
#106720=CARTESIAN_POINT('Ctrl Pts',(-19.5730414964587,21.1546302039879,
-10.2351567834308));
#106721=CARTESIAN_POINT('Ctrl Pts',(-19.5730886237369,21.1546098590378,
-10.2351537193111));
#106722=CARTESIAN_POINT('Ctrl Pts',(-19.5731812801373,21.154569855067,-10.2351476950012));
#106723=CARTESIAN_POINT('Ctrl Pts',(-19.5732268080293,21.1545501967129,
-10.2351447348902));
#106724=CARTESIAN_POINT('Ctrl Pts',(-19.5733163139483,21.1545115454851,
-10.2351389154559));
#106725=CARTESIAN_POINT('Ctrl Pts',(-19.5733603059771,21.1544925466917,
-10.2351360552213));
#106726=CARTESIAN_POINT('Ctrl Pts',(-19.5734468003774,21.1544551889559,
-10.2351304316238));
#106727=CARTESIAN_POINT('Ctrl Pts',(-19.573489302699,21.1544368301536,-10.2351276682632));
#106728=CARTESIAN_POINT('Ctrl Pts',(-19.5735728760549,21.1544007275378,
-10.2351222346163));
#106729=CARTESIAN_POINT('Ctrl Pts',(-19.5736139471291,21.1543829838166,
-10.2351195643269));
#106730=CARTESIAN_POINT('Ctrl Pts',(-19.573694709497,21.1543480894354,-10.2351143134719));
#106731=CARTESIAN_POINT('Ctrl Pts',(-19.5737344009397,21.1543309388131,
-10.2351117328961));
#106732=CARTESIAN_POINT('Ctrl Pts',(-19.5738124537,21.1542972094759,-10.2351066582384));
#106733=CARTESIAN_POINT('Ctrl Pts',(-19.5738508149958,21.1542806308656,
-10.2351041641574));
#106734=CARTESIAN_POINT('Ctrl Pts',(-19.5806180562704,21.1513557927854,
-10.2346641894215));
#106735=CARTESIAN_POINT('Ctrl Pts',(-19.5873318495993,21.1484125766935,
-10.2342279027148));
#106736=CARTESIAN_POINT('Ctrl Pts',(-19.6058483423217,21.1401803287857,
-10.2330251381579));
#106737=CARTESIAN_POINT('Ctrl Pts',(-19.6176181930145,21.1348178638103,
-10.2322611822493));
#106738=CARTESIAN_POINT('Ctrl Pts',(-19.6437523370135,21.1226204396081,
-10.2305657146303));
#106739=CARTESIAN_POINT('Ctrl Pts',(-19.6580903071511,21.1157307274413,
-10.2296361073986));
#106740=CARTESIAN_POINT('Ctrl Pts',(-19.702145179987,21.0939468272331,-10.2267802678017));
#106741=CARTESIAN_POINT('Ctrl Pts',(-19.7315907130382,21.0785135283598,
-10.2248722292976));
#106742=CARTESIAN_POINT('Ctrl Pts',(-19.8455660918575,21.0153102069606,
-10.2174706515384));
#106743=CARTESIAN_POINT('Ctrl Pts',(-19.9271357089285,20.962440507687,-10.212144414821));
#106744=CARTESIAN_POINT('Ctrl Pts',(-20.1322479364308,20.8084942117171,
-10.198190740769));
#106745=CARTESIAN_POINT('Ctrl Pts',(-20.2484750443433,20.6987617478178,
-10.1896972785582));
#106746=CARTESIAN_POINT('Ctrl Pts',(-20.3605847917494,20.5660346882025,
-10.1794909032523));
#106747=CARTESIAN_POINT('Ctrl Pts',(-20.3697800014617,20.5549199575445,
-10.1786364442597));
#106748=CARTESIAN_POINT('Ctrl Pts',(-20.3823824722885,20.5393657337455,
-10.1774396334951));
#106749=CARTESIAN_POINT('Ctrl Pts',(-20.3858870313162,20.5350051101431,
-10.1771039938543));
#106750=CARTESIAN_POINT('Ctrl Pts',(-20.3914768025684,20.5279931762741,
-10.1765640059058));
#106751=CARTESIAN_POINT('Ctrl Pts',(-20.3935730619795,20.5253506491755,
-10.1763604430214));
#106752=CARTESIAN_POINT('Ctrl Pts',(-20.3979316711108,20.5198291716477,
-10.1759349485047));
#106753=CARTESIAN_POINT('Ctrl Pts',(-20.4001928675041,20.5169493612755,
-10.1757129347041));
#106754=CARTESIAN_POINT('Ctrl Pts',(-20.405633105068,20.5099836654563,-10.1751757362406));
#106755=CARTESIAN_POINT('Ctrl Pts',(-20.4088046410741,20.5058919700169,
-10.1748600254042));
#106756=CARTESIAN_POINT('Ctrl Pts',(-20.4197880307085,20.4916141102361,
-10.173757939017));
#106757=CARTESIAN_POINT('Ctrl Pts',(-20.4275220388204,20.4813687926063,
-10.1729663755848));
#106758=CARTESIAN_POINT('Ctrl Pts',(-20.4722134396685,20.4210322383863,
-10.1683034958164));
#106759=CARTESIAN_POINT('Ctrl Pts',(-20.5070370476685,20.369405002454,-10.164309539088));
#106760=CARTESIAN_POINT('Ctrl Pts',(-20.6118061721582,20.1982660253265,
-10.1512361186923));
#106761=CARTESIAN_POINT('Ctrl Pts',(-20.6723278871939,20.0734026319898,
-10.1419706979438));
#106762=CARTESIAN_POINT('Ctrl Pts',(-20.7344247313902,19.9050267018588,
-10.130313183837));
#106763=CARTESIAN_POINT('Ctrl Pts',(-20.7474992329999,19.8661284610667,
-10.1276721286586));
#106764=CARTESIAN_POINT('Ctrl Pts',(-20.7623061626206,19.8174325798067,
-10.1244342720389));
#106765=CARTESIAN_POINT('Ctrl Pts',(-20.7651107253494,19.8079720170767,
-10.1238083728947));
#106766=CARTESIAN_POINT('Ctrl Pts',(-20.783378684374,19.744729851012,-10.119645452622));
#106767=CARTESIAN_POINT('Ctrl Pts',(-20.7967715207409,19.6903695042325,
-10.116169605456));
#106768=CARTESIAN_POINT('Ctrl Pts',(-20.8104072878551,19.6237546954499,
-10.112030509052));
#106769=CARTESIAN_POINT('Ctrl Pts',(-20.8127188525531,19.6119508761455,
-10.1113015747757));
#106770=CARTESIAN_POINT('Ctrl Pts',(-20.8163752070018,19.5923978742264,
-10.110101367228));
#106771=CARTESIAN_POINT('Ctrl Pts',(-20.8177776139856,19.5846598710808,
-10.1096282667333));
#106772=CARTESIAN_POINT('Ctrl Pts',(-20.8202374445089,19.5706426942465,
-10.1087745941513));
#106773=CARTESIAN_POINT('Ctrl Pts',(-20.8213097124377,19.5643662521112,
-10.108393554067));
#106774=CARTESIAN_POINT('Ctrl Pts',(-20.8233364562906,19.5521716664567,
-10.107655532389));
#106775=CARTESIAN_POINT('Ctrl Pts',(-20.8242941435062,19.5462541250107,
-10.1072984522392));
#106776=CARTESIAN_POINT('Ctrl Pts',(-20.8263396723343,19.5332652342932,
-10.106516937583));
#106777=CARTESIAN_POINT('Ctrl Pts',(-20.8274168308279,19.5261922587443,
-10.1060928441082));
#106778=CARTESIAN_POINT('Ctrl Pts',(-20.8299772003143,19.508787698909,-10.1050528142087));
#106779=CARTESIAN_POINT('Ctrl Pts',(-20.8314199105171,19.4984502785485,
-10.104438153699));
#106780=CARTESIAN_POINT('Ctrl Pts',(-20.8449846038358,19.3957107033154,
-10.0983586071851));
#106781=CARTESIAN_POINT('Ctrl Pts',(-20.8510696179301,19.3026105798559,
-10.0930912443828));
#106782=CARTESIAN_POINT('Ctrl Pts',(-20.8509993992227,19.2094051048361,
-10.0879365117025));
#106783=CARTESIAN_POINT('Ctrl Pts',(-20.8509994011045,19.2094076046327,
-10.0879366499539));
#106784=CARTESIAN_POINT('Ctrl Pts',(-20.8508903570022,19.0644396499636,
-10.0799191880673));
#106785=CARTESIAN_POINT('Ctrl Pts',(-20.8358914557206,18.9198677623656,
-10.0722246121862));
#106786=CARTESIAN_POINT('Ctrl Pts',(-20.7926402107778,18.7128956226968,
-10.0604947085716));
#106787=CARTESIAN_POINT('Ctrl Pts',(-20.775987532445,18.6485120637171,-10.056735705653));
#106788=CARTESIAN_POINT('Ctrl Pts',(-20.7524080825635,18.5723339612825,
-10.0520405686672));
#106789=CARTESIAN_POINT('Ctrl Pts',(-20.7483605188363,18.5596804342305,
-10.0512523078793));
#106790=CARTESIAN_POINT('Ctrl Pts',(-20.7425481579392,18.5420823325455,
-10.0501432138957));
#106791=CARTESIAN_POINT('Ctrl Pts',(-20.7408835587576,18.5371046603246,
-10.0498280660244));
#106792=CARTESIAN_POINT('Ctrl Pts',(-20.7380219448138,18.5286521768047,
-10.0492903910603));
#106793=CARTESIAN_POINT('Ctrl Pts',(-20.7368343465263,18.5251741567682,
-10.0490684186571));
#106794=CARTESIAN_POINT('Ctrl Pts',(-20.7345445654253,18.5185249368981,
-10.0486426263969));
#106795=CARTESIAN_POINT('Ctrl Pts',(-20.7334438884132,18.5153532448196,
-10.0484389005606));
#106796=CARTESIAN_POINT('Ctrl Pts',(-20.7305162333362,18.5069813137827,
-10.0478995311231));
#106797=CARTESIAN_POINT('Ctrl Pts',(-20.7286764970099,18.5017856098278,
-10.0475631397474));
#106798=CARTESIAN_POINT('Ctrl Pts',(-20.7254160069984,18.4926905187973,
-10.0469714583051));
#106799=CARTESIAN_POINT('Ctrl Pts',(-20.7240040333705,18.4887880020968,
-10.0467166641269));
#106800=CARTESIAN_POINT('Ctrl Pts',(-20.7225806138021,18.4848897174598,
-10.0464612475213));
#106801=CARTESIAN_POINT('Origin',(-18.734,19.211,0.));
#106802=CARTESIAN_POINT('',(-20.7225807588464,18.4848901146894,-9.24346988827878));
#106803=CARTESIAN_POINT('',(-20.7225806137986,18.4848897174502,-9.46634970542581));
#106804=CARTESIAN_POINT('',(-20.7225806137986,18.4848897174502,0.));
#106805=CARTESIAN_POINT('',(-20.8516085051224,19.2128934567755,-9.51094371951089));
#106806=CARTESIAN_POINT('Ctrl Pts',(-20.7225806137986,18.4848897174502,
-9.46634970542581));
#106807=CARTESIAN_POINT('Ctrl Pts',(-20.7472616943129,18.5524831938379,
-9.47066129020357));
#106808=CARTESIAN_POINT('Ctrl Pts',(-20.768494307004,18.6213418962955,-9.47497287498133));
#106809=CARTESIAN_POINT('Ctrl Pts',(-20.7861614183071,18.6910745118658,
-9.4792844597591));
#106810=CARTESIAN_POINT('Ctrl Pts',(-20.8038310812988,18.7608171990267,
-9.48359666726579));
#106811=CARTESIAN_POINT('Ctrl Pts',(-20.8179341108459,18.8314335643017,
-9.48790887477247));
#106812=CARTESIAN_POINT('Ctrl Pts',(-20.8284043874146,18.902521050996,-9.49222108227916));
#106813=CARTESIAN_POINT('Ctrl Pts',(-20.8388856923757,18.9736834144808,
-9.49653783185468));
#106814=CARTESIAN_POINT('Ctrl Pts',(-20.8457265542653,19.0453173949163,
-9.50085458143021));
#106815=CARTESIAN_POINT('Ctrl Pts',(-20.8489127423905,19.1170154689625,
-9.50517133100573));
#106816=CARTESIAN_POINT('Ctrl Pts',(-20.8503329346207,19.1489737349782,
-9.50709545286107));
#106817=CARTESIAN_POINT('Ctrl Pts',(-20.8510277144022,19.1809447313957,
-9.5090195747164));
#106818=CARTESIAN_POINT('Ctrl Pts',(-20.8509991540684,19.2128925310398,
-9.51094369657173));
#106819=CARTESIAN_POINT('Ctrl Pts',(-20.8516474640139,19.2128935159625,
-9.51094372097751));
#106820=CARTESIAN_POINT('Ctrl Pts',(-20.8529701716602,19.3558822341492,
-9.51955279572482));
#106821=CARTESIAN_POINT('Ctrl Pts',(-20.77452049264,20.2015184074521,-9.57055380603263));
#106822=CARTESIAN_POINT('Ctrl Pts',(-19.6371491634786,21.5456631571965,
-9.66394675190087));
#106823=CARTESIAN_POINT('Ctrl Pts',(-17.2597752658646,21.2341144066337,
-9.79112255858231));
#106824=CARTESIAN_POINT('Ctrl Pts',(-16.2349110611132,19.0664837566253,
-9.91829836526376));
#106825=CARTESIAN_POINT('Ctrl Pts',(-17.5028058468379,17.031437790224,-10.0454741719452));
#106826=CARTESIAN_POINT('Ctrl Pts',(-19.6892758366696,16.9991228861485,
-10.1614588056287));
#106827=CARTESIAN_POINT('Ctrl Pts',(-20.5391741505579,17.9993261502973,
-10.2350515037519));
#106828=CARTESIAN_POINT('Ctrl Pts',(-20.7219730443073,18.4851210911022,
-10.2662522663145));
#106829=CARTESIAN_POINT('Ctrl Pts',(-20.7225806138021,18.4848897174598,
-10.0464612475213));
#106830=CARTESIAN_POINT('Ctrl Pts',(-20.7192292584429,18.4757114418486,
-10.0458598845578));
#106831=CARTESIAN_POINT('Ctrl Pts',(-20.7158144538027,18.4665566261871,
-10.0452550715018));
#106832=CARTESIAN_POINT('Ctrl Pts',(-20.6531107477152,18.3019423801365,
-10.0342938815402));
#106833=CARTESIAN_POINT('Ctrl Pts',(-20.5757664518257,18.1539936132858,
-10.0231064405996));
#106834=CARTESIAN_POINT('Ctrl Pts',(-20.4366046550753,17.9503358154075,
-10.0069020249956));
#106835=CARTESIAN_POINT('Ctrl Pts',(-20.3875635364868,17.8866637597059,
-10.0016903281187));
#106836=CARTESIAN_POINT('Ctrl Pts',(-20.3092873850567,17.7961835956228,
-9.99410986078368));
#106837=CARTESIAN_POINT('Ctrl Pts',(-20.2827305771936,17.7671614645455,
-9.99164823551441));
#106838=CARTESIAN_POINT('Ctrl Pts',(-20.2369236068718,17.7198212613663,
-9.98758111794582));
#106839=CARTESIAN_POINT('Ctrl Pts',(-20.2181103780658,17.7010960676583,
-9.98595788160913));
#106840=CARTESIAN_POINT('Ctrl Pts',(-20.1918823896307,17.6759547994022,
-9.98375726203708));
#106841=CARTESIAN_POINT('Ctrl Pts',(-20.1847684802612,17.6692297020659,
-9.98316646069937));
#106842=CARTESIAN_POINT('Ctrl Pts',(-20.1732499953931,17.6584910783321,
-9.98221949472933));
#106843=CARTESIAN_POINT('Ctrl Pts',(-20.1688747389153,17.6544464397751,
-9.98186199598629));
#106844=CARTESIAN_POINT('Ctrl Pts',(-20.1597234017734,17.6460580012073,
-9.98111879015933));
#106845=CARTESIAN_POINT('Ctrl Pts',(-20.1549444041178,17.6417174633672,
-9.98073322400363));
#106846=CARTESIAN_POINT('Ctrl Pts',(-20.1438651652245,17.6317468206085,
-9.97984517530119));
#106847=CARTESIAN_POINT('Ctrl Pts',(-20.1375508973816,17.6261324123611,
-9.97934335703039));
#106848=CARTESIAN_POINT('Ctrl Pts',(-20.1204817236984,17.611137165082,-9.97799816822268));
#106849=CARTESIAN_POINT('Ctrl Pts',(-20.1096651777285,17.6018269221928,
-9.97715772927185));
#106850=CARTESIAN_POINT('Ctrl Pts',(-20.0094118528506,17.517284481492,-9.96947482119003));
#106851=CARTESIAN_POINT('Ctrl Pts',(-19.9139779331128,17.4494651585837,
-9.96294926674155));
#106852=CARTESIAN_POINT('Ctrl Pts',(-19.6733869540662,17.3068623850346,
-9.9476384555831));
#106853=CARTESIAN_POINT('Ctrl Pts',(-19.524263822558,17.2402998388123,-9.93903632368726));
#106854=CARTESIAN_POINT('Ctrl Pts',(-19.3380437823101,17.1817455077592,
-9.92782714614726));
#106855=CARTESIAN_POINT('Ctrl Pts',(-19.3068600295617,17.1727228324961,
-9.92593382656331));
#106856=CARTESIAN_POINT('Ctrl Pts',(-19.2684875435943,17.1625702525105,
-9.9235704599097));
#106857=CARTESIAN_POINT('Ctrl Pts',(-19.2614825854748,17.1607552625992,
-9.92313766635831));
#106858=CARTESIAN_POINT('Ctrl Pts',(-19.250485711119,17.1579660514445,-9.92245591419394));
#106859=CARTESIAN_POINT('Ctrl Pts',(-19.2464999533063,17.156967458653,-9.92220833976146));
#106860=CARTESIAN_POINT('Ctrl Pts',(-19.2390438849293,17.1551224662386,
-9.92174427360243));
#106861=CARTESIAN_POINT('Ctrl Pts',(-19.2355743308113,17.1542732438305,
-9.92152794697672));
#106862=CARTESIAN_POINT('Ctrl Pts',(-19.2276487042941,17.1523545820157,
-9.92103292316839));
#106863=CARTESIAN_POINT('Ctrl Pts',(-19.223191313764,17.1512908317278,-9.92075390373884));
#106864=CARTESIAN_POINT('Ctrl Pts',(-19.2094772777523,17.1480650231234,
-9.91989362591211));
#106865=CARTESIAN_POINT('Ctrl Pts',(-19.2002096443159,17.1459508673444,
-9.91930972473851));
#106866=CARTESIAN_POINT('Ctrl Pts',(-19.1166677079326,17.1274840974736,
-9.91402529553097));
#106867=CARTESIAN_POINT('Ctrl Pts',(-19.0415842745261,17.1150843416033,
-9.90912895176016));
#106868=CARTESIAN_POINT('Ctrl Pts',(-18.8155315308582,17.0901606878071,
-9.8942539240383));
#106869=CARTESIAN_POINT('Ctrl Pts',(-18.663693402277,17.0897572228357,-9.88412220250481));
#106870=CARTESIAN_POINT('Ctrl Pts',(-18.4580374486812,17.1113333495289,
-9.87082768138821));
#106871=CARTESIAN_POINT('Ctrl Pts',(-18.4032094151102,17.1192701430802,
-9.867320486863));
#106872=CARTESIAN_POINT('Ctrl Pts',(-18.3148993658855,17.1356135548935,
-9.86173753465641));
#106873=CARTESIAN_POINT('Ctrl Pts',(-18.2812033465313,17.142703684837,-9.85962289906963));
#106874=CARTESIAN_POINT('Ctrl Pts',(-18.2371603710423,17.1530990030193,
-9.85687790975412));
#106875=CARTESIAN_POINT('Ctrl Pts',(-18.2266461872596,17.1556659040956,
-9.85622403382406));
#106876=CARTESIAN_POINT('Ctrl Pts',(-18.2094605105504,17.1600014749622,
-9.85515747661951));
#106877=CARTESIAN_POINT('Ctrl Pts',(-18.2027772598948,17.1617223155832,
-9.85474326003886));
#106878=CARTESIAN_POINT('Ctrl Pts',(-18.1898588556673,17.1651160618714,
-9.85394362566391));
#106879=CARTESIAN_POINT('Ctrl Pts',(-18.1836227126032,17.1667848654824,
-9.85355808020826));
#106880=CARTESIAN_POINT('Ctrl Pts',(-18.1692444773468,17.1707030729017,
-9.85267018338997));
#106881=CARTESIAN_POINT('Ctrl Pts',(-18.1611079849665,17.1729727446965,
-9.85216849557217));
#106882=CARTESIAN_POINT('Ctrl Pts',(-18.1392696098283,17.1792056687413,
-9.85082388737276));
#106883=CARTESIAN_POINT('Ctrl Pts',(-18.1255936861256,17.1832588395962,
-9.84998389456965));
#106884=CARTESIAN_POINT('Ctrl Pts',(-18.0001577331489,17.2218179266526,
-9.84229581169312));
#106885=CARTESIAN_POINT('Ctrl Pts',(-17.8913895626666,17.2653939960854,
-9.83576520565507));
#106886=CARTESIAN_POINT('Ctrl Pts',(-17.6409649188848,17.3906861326746,
-9.82043611232572));
#106887=CARTESIAN_POINT('Ctrl Pts',(-17.5040963052504,17.4802217977321,
-9.81182142397062));
#106888=CARTESIAN_POINT('Ctrl Pts',(-17.3541557404107,17.6051501542586,
-9.80061117768796));
#106889=CARTESIAN_POINT('Ctrl Pts',(-17.3299143814775,17.6263021644634,
-9.79873437698213));
#106890=CARTESIAN_POINT('Ctrl Pts',(-17.3008379550254,17.6528640532562,
-9.79638939059324));
#106891=CARTESIAN_POINT('Ctrl Pts',(-17.2955350581716,17.6577583306483,
-9.79595777837437));
#106892=CARTESIAN_POINT('Ctrl Pts',(-17.2872553878152,17.6654787692485,
-9.79527747772444));
#106893=CARTESIAN_POINT('Ctrl Pts',(-17.2842615769759,17.6682866916569,
-9.79503016376186));
#106894=CARTESIAN_POINT('Ctrl Pts',(-17.2786772207057,17.6735549205963,
-9.79456631734594));
#106895=CARTESIAN_POINT('Ctrl Pts',(-17.2760847308732,17.6760130842573,
-9.79434994835765));
#106896=CARTESIAN_POINT('Ctrl Pts',(-17.2701762540741,17.6816438929165,
-9.79385447278043));
#106897=CARTESIAN_POINT('Ctrl Pts',(-17.2668643645917,17.6848207550195,
-9.7935750416618));
#106898=CARTESIAN_POINT('Ctrl Pts',(-17.2582424576261,17.6931451420628,
-9.79284320079083));
#106899=CARTESIAN_POINT('Ctrl Pts',(-17.2529490907731,17.6983097163529,
-9.79238950999087));
#106900=CARTESIAN_POINT('Ctrl Pts',(-17.2183372667072,17.7324352258961,
-9.78939468194003));
#106901=CARTESIAN_POINT('Ctrl Pts',(-17.1898448105618,17.7622172187049,
-9.78679518565037));
#106902=CARTESIAN_POINT('Ctrl Pts',(-17.147220574699,17.8094569786565,-9.78271912947184));
#106903=CARTESIAN_POINT('Ctrl Pts',(-17.1324652284145,17.826341882549,-9.78127101771809));
#106904=CARTESIAN_POINT('Ctrl Pts',(-17.0165750514617,17.9632887680826,
-9.76961529082282));
#106905=CARTESIAN_POINT('Ctrl Pts',(-16.9288089313468,18.0940295422687,
-9.7590752129637));
#106906=CARTESIAN_POINT('Ctrl Pts',(-16.8280505717015,18.2875352114421,
-9.7449863694245));
#106907=CARTESIAN_POINT('Ctrl Pts',(-16.8021637192357,18.3429907133462,
-9.74109728006499));
#106908=CARTESIAN_POINT('Ctrl Pts',(-16.7645366432666,18.4336514308909,
-9.73498231498705));
#106909=CARTESIAN_POINT('Ctrl Pts',(-16.7512570201627,18.4681761595308,
-9.73270769071316));
#106910=CARTESIAN_POINT('Ctrl Pts',(-16.7351741821253,18.5134989736038,
-9.72978928421131));
#106911=CARTESIAN_POINT('Ctrl Pts',(-16.7315426414751,18.5239942746394,
-9.72911810615832));
#106912=CARTESIAN_POINT('Ctrl Pts',(-16.7257686508755,18.5411161758072,
-9.72803054424939));
#106913=CARTESIAN_POINT('Ctrl Pts',(-16.7235760491618,18.5477255249743,
-9.72761250700058));
#106914=CARTESIAN_POINT('Ctrl Pts',(-16.7194207240301,18.5604612060101,
-9.72681035980897));
#106915=CARTESIAN_POINT('Ctrl Pts',(-16.7174532386901,18.5665858920584,
-9.72642609656468));
#106916=CARTESIAN_POINT('Ctrl Pts',(-16.7130102760682,18.5806362340416,
-9.72554795302985));
#106917=CARTESIAN_POINT('Ctrl Pts',(-16.7105534385819,18.588567708297,-9.72505468926941));
#106918=CARTESIAN_POINT('Ctrl Pts',(-16.7041462558614,18.6096910925134,
-9.72374739360048));
#106919=CARTESIAN_POINT('Ctrl Pts',(-16.7002778116199,18.6229075764203,
-9.72293603741057));
#106920=CARTESIAN_POINT('Ctrl Pts',(-16.6715227363951,18.7248271891946,
-9.71672789116723));
#106921=CARTESIAN_POINT('Ctrl Pts',(-16.6523196348054,18.815037454539,-9.71152165510277));
#106922=CARTESIAN_POINT('Ctrl Pts',(-16.6187969411326,19.0454611850514,
-9.69864331870203));
#106923=CARTESIAN_POINT('Ctrl Pts',(-16.6124727143517,19.1863666960421,
-9.69116392748577));
#106924=CARTESIAN_POINT('Ctrl Pts',(-16.6230746347889,19.3798061231709,
-9.6804441511693));
#106925=CARTESIAN_POINT('Ctrl Pts',(-16.6279653658204,19.4326275173585,
-9.6774669403305));
#106926=CARTESIAN_POINT('Ctrl Pts',(-16.638421692189,19.5126753421487,-9.67280613148938));
#106927=CARTESIAN_POINT('Ctrl Pts',(-16.6425486019467,19.5400704172097,
-9.67118414829697));
#106928=CARTESIAN_POINT('Ctrl Pts',(-16.6483699305577,19.5741577611718,
-9.66912348596524));
#106929=CARTESIAN_POINT('Ctrl Pts',(-16.6495612934932,19.5809346184253,
-9.66871170314222));
#106930=CARTESIAN_POINT('Ctrl Pts',(-16.6515028342518,19.5916715102366,
-9.66805578327073));
#106931=CARTESIAN_POINT('Ctrl Pts',(-16.6522313320841,19.5956354855115,
-9.66781286204611));
#106932=CARTESIAN_POINT('Ctrl Pts',(-16.6536294726477,19.6031228528446,
-9.66735253984719));
#106933=CARTESIAN_POINT('Ctrl Pts',(-16.6542967508952,19.6066466324067,
-9.66713527412185));
#106934=CARTESIAN_POINT('Ctrl Pts',(-16.655846612084,19.6147189173539,-9.66663614374831));
#106935=CARTESIAN_POINT('Ctrl Pts',(-16.6567351748868,19.6192662285108,
-9.66635394171129));
#106936=CARTESIAN_POINT('Ctrl Pts',(-16.6591420175153,19.6313722058962,
-9.66559997756064));
#106937=CARTESIAN_POINT('Ctrl Pts',(-16.6606866560881,19.6389254757344,
-9.66512677221462));
#106938=CARTESIAN_POINT('Ctrl Pts',(-16.6720299713919,19.6928907500064,
-9.66172678035979));
#106939=CARTESIAN_POINT('Ctrl Pts',(-16.6833441228806,19.7389666757993,
-9.65872275899436));
#106940=CARTESIAN_POINT('Ctrl Pts',(-16.7061569268642,19.8200100078691,
-9.6533034696357));
#106941=CARTESIAN_POINT('Ctrl Pts',(-16.7170387987474,19.8551335458005,
-9.65090847010828));
#106942=CARTESIAN_POINT('Ctrl Pts',(-16.7290822194177,19.8907016370013,
-9.6484462209914));
#106943=CARTESIAN_POINT('Ctrl Pts',(-16.7293356236529,19.8914486464457,
-9.64839449140688));
#106944=CARTESIAN_POINT('Ctrl Pts',(-16.7712938712655,20.014910343315,-9.63984213495151));
#106945=CARTESIAN_POINT('Ctrl Pts',(-16.8241832259323,20.133545787856,-9.63119483620107));
#106946=CARTESIAN_POINT('Ctrl Pts',(-16.9306698863168,20.3234047045237,
-9.61710172206642));
#106947=CARTESIAN_POINT('Ctrl Pts',(-16.9785020373741,20.3974543903341,
-9.61152620200881));
#106948=CARTESIAN_POINT('Ctrl Pts',(-17.0429888147084,20.4848093974725,
-9.60486274947755));
#106949=CARTESIAN_POINT('Ctrl Pts',(-17.0554027018575,20.5011241672537,
-9.60361401279766));
#106950=CARTESIAN_POINT('Ctrl Pts',(-17.0735168984427,20.5242262992094,
-9.60183908637065));
#106951=CARTESIAN_POINT('Ctrl Pts',(-17.0790255955911,20.5311617961332,
-9.60130535176057));
#106952=CARTESIAN_POINT('Ctrl Pts',(-17.0886517344082,20.5431262413686,
-9.60038299268831));
#106953=CARTESIAN_POINT('Ctrl Pts',(-17.0927490778357,20.5481711371344,
-9.59999356997746));
#106954=CARTESIAN_POINT('Ctrl Pts',(-17.1006725612993,20.5578357200678,
-9.59924653930038));
#106955=CARTESIAN_POINT('Ctrl Pts',(-17.1044952253837,20.5624581641716,
-9.59888879617962));
#106956=CARTESIAN_POINT('Ctrl Pts',(-17.1145622903182,20.5745266548548,
-9.59795356289297));
#106957=CARTESIAN_POINT('Ctrl Pts',(-17.1208384511196,20.5819461171163,
-9.59737737356893));
#106958=CARTESIAN_POINT('Ctrl Pts',(-17.142805149784,20.6075546780837,-9.59538407980322));
#106959=CARTESIAN_POINT('Ctrl Pts',(-17.158754372078,20.6255201664292,-9.59397766381086));
#106960=CARTESIAN_POINT('Ctrl Pts',(-17.2751770633516,20.7522488723551,
-9.58398811811653));
#106961=CARTESIAN_POINT('Ctrl Pts',(-17.3865124199935,20.8504805127702,
-9.57591395001439));
#106962=CARTESIAN_POINT('Ctrl Pts',(-17.5448576694999,20.9630743684982,
-9.56536229977445));
#106963=CARTESIAN_POINT('Ctrl Pts',(-17.5833811467825,20.9886108206187,
-9.56285552616156));
#106964=CARTESIAN_POINT('Ctrl Pts',(-17.6834747591274,21.0503430218408,
-9.55642254511744));
#106965=CARTESIAN_POINT('Ctrl Pts',(-17.7460932155647,21.0847194742361,
-9.55247223031956));
#106966=CARTESIAN_POINT('Ctrl Pts',(-17.8405323244734,21.1305134029403,
-9.54645283652381));
#106967=CARTESIAN_POINT('Ctrl Pts',(-17.8710840248494,21.1444404374242,
-9.5444962879679));
#106968=CARTESIAN_POINT('Ctrl Pts',(-17.9086746611854,21.1605077679038,
-9.54206261370465));
#106969=CARTESIAN_POINT('Ctrl Pts',(-17.9154121177493,21.163346364633,-9.54162540426563));
#106970=CARTESIAN_POINT('Ctrl Pts',(-17.9259740272493,21.1677319811952,
-9.5409382274285));
#106971=CARTESIAN_POINT('Ctrl Pts',(-17.9297886027342,21.1693028485686,
-9.54068968077592));
#106972=CARTESIAN_POINT('Ctrl Pts',(-17.936912541271,21.172212208473,-9.54022478487092));
#106973=CARTESIAN_POINT('Ctrl Pts',(-17.9402207066579,21.173553483691,-9.54000860679316));
#106974=CARTESIAN_POINT('Ctrl Pts',(-17.9477608243921,21.1765883944744,
-9.53951522564785));
#106975=CARTESIAN_POINT('Ctrl Pts',(-17.9519948472268,21.1782767263126,
-9.53923770867076));
#106976=CARTESIAN_POINT('Ctrl Pts',(-17.9630171687524,21.182630711101,-9.53851410512816));
#106977=CARTESIAN_POINT('Ctrl Pts',(-17.9698137820198,21.1852749574866,
-9.53806678319188));
#106978=CARTESIAN_POINT('Ctrl Pts',(-18.0131748559959,21.2018872853939,
-9.53520638856773));
#106979=CARTESIAN_POINT('Ctrl Pts',(-18.0501046568233,21.2148731954422,
-9.53274068511487));
#106980=CARTESIAN_POINT('Ctrl Pts',(-18.0991255561503,21.230597941644,-9.52944826186314));
#106981=CARTESIAN_POINT('Ctrl Pts',(-18.1109133790197,21.234265790091,-9.52865508276562));
#106982=CARTESIAN_POINT('Ctrl Pts',(-18.1458487131312,21.2448018662563,
-9.52630129409243));
#106983=CARTESIAN_POINT('Ctrl Pts',(-18.1690820104827,21.2513773108174,
-9.52473200362552));
#106984=CARTESIAN_POINT('Ctrl Pts',(-18.3317803462426,21.294432047482,-9.51373625927888));
#106985=CARTESIAN_POINT('Ctrl Pts',(-18.4745551729318,21.3169827093222,
-9.50408913664737));
#106986=CARTESIAN_POINT('Ctrl Pts',(-18.68023113681,21.3282194912357,-9.49078088416227));
#106987=CARTESIAN_POINT('Ctrl Pts',(-18.7420711405565,21.3288870253313,
-9.48684929269609));
#106988=CARTESIAN_POINT('Ctrl Pts',(-18.8410951737027,21.3256176609582,
-9.48067566997719));
#106989=CARTESIAN_POINT('Ctrl Pts',(-18.8782965760856,21.3234052648851,
-9.47838372291228));
#106990=CARTESIAN_POINT('Ctrl Pts',(-18.9265161329777,21.3192576990847,
-9.47544662757999));
#106991=CARTESIAN_POINT('Ctrl Pts',(-18.9376025842254,21.3182159315848,
-9.47477364703566));
#106992=CARTESIAN_POINT('Ctrl Pts',(-18.9556144879361,21.3163799179574,
-9.47368389618655));
#106993=CARTESIAN_POINT('Ctrl Pts',(-18.9625450378592,21.3156388639573,
-9.47326546000194));
#106994=CARTESIAN_POINT('Ctrl Pts',(-18.9758627018832,21.3141483038161,
-9.4724630360659));
#106995=CARTESIAN_POINT('Ctrl Pts',(-18.9822502983172,21.3134038967813,
-9.47207889239622));
#106996=CARTESIAN_POINT('Ctrl Pts',(-18.9968632875222,21.3116333806082,
-9.4712016990185));
#106997=CARTESIAN_POINT('Ctrl Pts',(-19.0050862775266,21.310588040729,-9.47070926125003));
#106998=CARTESIAN_POINT('Ctrl Pts',(-19.0269054865848,21.3076839726392,
-9.46940560537363));
#106999=CARTESIAN_POINT('Ctrl Pts',(-19.0404902736747,21.3057412801023,
-9.46859703901192));
#107000=CARTESIAN_POINT('Ctrl Pts',(-19.1432879196679,21.2900192595542,
-9.46250020157523));
#107001=CARTESIAN_POINT('Ctrl Pts',(-19.2315620229315,21.2706777856789,
-9.4573944194948));
#107002=CARTESIAN_POINT('Ctrl Pts',(-19.4524107508922,21.2072545595245,
-9.44467444557782));
#107003=CARTESIAN_POINT('Ctrl Pts',(-19.5823414692185,21.1555979458743,
-9.43725498332676));
#107004=CARTESIAN_POINT('Ctrl Pts',(-19.7553604313235,21.0661466388808,
-9.42649624725405));
#107005=CARTESIAN_POINT('Ctrl Pts',(-19.8034593809973,21.0388407930322,
-9.42339814111303));
#107006=CARTESIAN_POINT('Ctrl Pts',(-19.8746319785227,20.9946644931094,
-9.41856625612374));
#107007=CARTESIAN_POINT('Ctrl Pts',(-19.8985260773497,20.9791569980145,
-9.41689961041943));
#107008=CARTESIAN_POINT('Ctrl Pts',(-19.9278456881352,20.9592762042554,
-9.41478899006835));
#107009=CARTESIAN_POINT('Ctrl Pts',(-19.9335733775351,20.9553511465029,
-9.41437349798387));
#107010=CARTESIAN_POINT('Ctrl Pts',(-19.9426064189659,20.9490954750897,
-9.4137130155325));
#107011=CARTESIAN_POINT('Ctrl Pts',(-19.9459246377392,20.9467834047782,
-9.41346927003957));
#107012=CARTESIAN_POINT('Ctrl Pts',(-19.9521703958111,20.9424048422397,
-9.41300831474008));
#107013=CARTESIAN_POINT('Ctrl Pts',(-19.9550993207377,20.9403404202584,
-9.41279124557676));
#107014=CARTESIAN_POINT('Ctrl Pts',(-19.961783870699,20.935603436798,-9.4122937769743));
#107015=CARTESIAN_POINT('Ctrl Pts',(-19.965536013193,20.9329260421533,-9.41201304812349));
#107016=CARTESIAN_POINT('Ctrl Pts',(-19.9754745491542,20.9257851580766,
-9.4112655599105));
#107017=CARTESIAN_POINT('Ctrl Pts',(-19.9816455459255,20.9213004947281,
-9.41079739545133));
#107018=CARTESIAN_POINT('Ctrl Pts',(-20.0247025304064,20.889652555765,-9.40750326036925));
#107019=CARTESIAN_POINT('Ctrl Pts',(-20.0607197777586,20.8613337140389,
-9.40460522594295));
#107020=CARTESIAN_POINT('Ctrl Pts',(-20.1245701421479,20.8076893628077,
-9.39924379076558));
#107021=CARTESIAN_POINT('Ctrl Pts',(-20.1527027882546,20.782745658247,-9.3967964306359));
#107022=CARTESIAN_POINT('Ctrl Pts',(-20.2758192823856,20.6675853647251,
-9.38574631474252));
#107023=CARTESIAN_POINT('Ctrl Pts',(-20.3629792372826,20.5694100832347,
-9.37700311419997));
#107024=CARTESIAN_POINT('Ctrl Pts',(-20.492797290268,20.3925790132671,-9.3627986467188));
#107025=CARTESIAN_POINT('Ctrl Pts',(-20.5405828338921,20.3181399016093,
-9.35720324779837));
#107026=CARTESIAN_POINT('Ctrl Pts',(-20.5935715870133,20.2229803661569,
-9.3505187402978));
#107027=CARTESIAN_POINT('Ctrl Pts',(-20.6033012793282,20.2048931142049,
-9.34926768696914));
#107028=CARTESIAN_POINT('Ctrl Pts',(-20.6168513889154,20.1788007058475,
-9.34749007724529));
#107029=CARTESIAN_POINT('Ctrl Pts',(-20.6208868697482,20.1709091120963,
-9.34695594462113));
#107030=CARTESIAN_POINT('Ctrl Pts',(-20.6277957962641,20.1571864165471,
-9.34603311890173));
#107031=CARTESIAN_POINT('Ctrl Pts',(-20.6306921430164,20.1513670394523,
-9.34564362532734));
#107032=CARTESIAN_POINT('Ctrl Pts',(-20.636208878151,20.140153563533,-9.34489661203854));
#107033=CARTESIAN_POINT('Ctrl Pts',(-20.6388332360916,20.1347614976619,
-9.34453895643853));
#107034=CARTESIAN_POINT('Ctrl Pts',(-20.6456466884508,20.1206099240407,
-9.34360429179119));
#107035=CARTESIAN_POINT('Ctrl Pts',(-20.6497985246213,20.1118325555888,
-9.34302858047085));
#107036=CARTESIAN_POINT('Ctrl Pts',(-20.6639911336504,20.0812861125865,
-9.34103860563081));
#107037=CARTESIAN_POINT('Ctrl Pts',(-20.6737226594694,20.0593747797715,
-9.33963498255815));
#107038=CARTESIAN_POINT('Ctrl Pts',(-20.742914465457,19.8961652662946,-9.32934412035894));
#107039=CARTESIAN_POINT('Ctrl Pts',(-20.7872440914993,19.7489445395367,
-9.32100728448304));
#107040=CARTESIAN_POINT('Ctrl Pts',(-20.8390879899929,19.4702807547455,
-9.30561476859398));
#107041=CARTESIAN_POINT('Ctrl Pts',(-20.8510398088518,19.3404434101152,
-9.29857236344691));
#107042=CARTESIAN_POINT('Ctrl Pts',(-20.8509988956986,19.2070755044686,
-9.29078137624927));
#107043=CARTESIAN_POINT('Ctrl Pts',(-20.8509902910738,19.2038004665512,
-9.29058970680201));
#107044=CARTESIAN_POINT('Ctrl Pts',(-20.8508966094021,19.1848667378393,
-9.28947952790844));
#107045=CARTESIAN_POINT('Ctrl Pts',(-20.850645400934,19.1692098497994,-9.28855320314594));
#107046=CARTESIAN_POINT('Ctrl Pts',(-20.8500635583701,19.1477742975099,
-9.28727189919378));
#107047=CARTESIAN_POINT('Ctrl Pts',(-20.8498828690298,19.14199162895,-9.28692493644138));
#107048=CARTESIAN_POINT('Ctrl Pts',(-20.8495580047971,19.1328018054636,
-9.28637136546238));
#107049=CARTESIAN_POINT('Ctrl Pts',(-20.8494292952819,19.1293940837142,
-9.28616561716021));
#107050=CARTESIAN_POINT('Ctrl Pts',(-20.8491463961677,19.1223550151953,
-9.2857396080172));
#107051=CARTESIAN_POINT('Ctrl Pts',(-20.8489910887203,19.1187237603298,
-9.28551928295103));
#107052=CARTESIAN_POINT('Ctrl Pts',(-20.8485986099401,19.1100692907856,
-9.28499286777946));
#107053=CARTESIAN_POINT('Ctrl Pts',(-20.8483528901894,19.1050465018352,
-9.28468630279956));
#107054=CARTESIAN_POINT('Ctrl Pts',(-20.847463120908,19.088096318964,-9.28364831690258));
#107055=CARTESIAN_POINT('Ctrl Pts',(-20.8467360342108,19.0761737677434,
-9.28291246841416));
#107056=CARTESIAN_POINT('Ctrl Pts',(-20.8368853576822,18.9344026989202,
-9.27409923509962));
#107057=CARTESIAN_POINT('Ctrl Pts',(-20.8159060912923,18.8056692574441,
-9.26548169761633));
#107058=CARTESIAN_POINT('Ctrl Pts',(-20.7661530760357,18.6137727633789,
-9.25238175885633));
#107059=CARTESIAN_POINT('Ctrl Pts',(-20.745904045056,18.5487650723614,-9.24789386380929));
#107060=CARTESIAN_POINT('Ctrl Pts',(-20.7225807588464,18.4848901146894,
-9.24346988827878));
#107061=CARTESIAN_POINT('Origin',(-18.734,19.211,0.));
#107062=CARTESIAN_POINT('',(-20.7225806137986,18.4848897174502,-8.44448866019381));
#107063=CARTESIAN_POINT('',(-20.7225805936643,18.484889662309,-8.66553669489169));
#107064=CARTESIAN_POINT('',(-20.7225806137986,18.4848897174502,0.));
#107065=CARTESIAN_POINT('',(-20.8509999986719,19.2110749873286,-8.71094372102529));
#107066=CARTESIAN_POINT('Ctrl Pts',(-20.7225805936643,18.484889662309,-8.66553669489169));
#107067=CARTESIAN_POINT('Ctrl Pts',(-20.7775649874159,18.6354740744751,
-8.67608256008694));
#107068=CARTESIAN_POINT('Ctrl Pts',(-20.8152928026166,18.7918910934345,
-8.68676276296178));
#107069=CARTESIAN_POINT('Ctrl Pts',(-20.8382408983242,18.9774167511052,
-8.69860361758393));
#107070=CARTESIAN_POINT('Ctrl Pts',(-20.8409993784059,19.0037691959386,
-8.70026806086961));
#107071=CARTESIAN_POINT('Ctrl Pts',(-20.8463154926722,19.0657772647298,
-8.70414334614212));
#107072=CARTESIAN_POINT('Ctrl Pts',(-20.8484662881568,19.1014603085863,
-8.70634148136337));
#107073=CARTESIAN_POINT('Ctrl Pts',(-20.8501018463908,19.1483376863317,
-8.70918910543019));
#107074=CARTESIAN_POINT('Ctrl Pts',(-20.8504028279016,19.1594959479233,
-8.70986396462703));
#107075=CARTESIAN_POINT('Ctrl Pts',(-20.8507477575,19.1775925090626,-8.71095377752203));
#107076=CARTESIAN_POINT('Ctrl Pts',(-20.8508458709025,19.1845294511023,
-8.71137042056006));
#107077=CARTESIAN_POINT('Ctrl Pts',(-20.8509497984104,19.1957925998922,
-8.71204512860756));
#107078=CARTESIAN_POINT('Ctrl Pts',(-20.8509764542535,19.2001185215261,
-8.71230384414341));
#107079=CARTESIAN_POINT('Ctrl Pts',(-20.8509965706163,19.2066147860699,
-8.7126917300085));
#107080=CARTESIAN_POINT('Ctrl Pts',(-20.850999953759,19.2087850666355,-8.71282121002485));
#107081=CARTESIAN_POINT('Ctrl Pts',(-20.8509999995292,19.2109553535338,
-8.71295058578666));
#107082=CARTESIAN_POINT('Ctrl Pts',(-20.8509999986719,19.2110749873286,
-8.71094372102529));
#107083=CARTESIAN_POINT('Ctrl Pts',(-20.8509972790728,19.2878531769888,
-8.71553605185449));
#107084=CARTESIAN_POINT('Ctrl Pts',(-20.8468134450972,19.3645459476709,
-8.7201283826837));
#107085=CARTESIAN_POINT('Ctrl Pts',(-20.8385019469854,19.440696658954,-8.72472071351291));
#107086=CARTESIAN_POINT('Ctrl Pts',(-20.8301661890788,19.5170696407114,
-8.72932644854457));
#107087=CARTESIAN_POINT('Ctrl Pts',(-20.8176787337246,19.5928969954346,
-8.73393218357623));
#107088=CARTESIAN_POINT('Ctrl Pts',(-20.8011445449252,19.6677301505114,
-8.7385379186079));
#107089=CARTESIAN_POINT('Ctrl Pts',(-20.7845848825973,19.742678597879,-8.74315074950159));
#107090=CARTESIAN_POINT('Ctrl Pts',(-20.7639661648764,19.8166294002047,
-8.74776358039528));
#107091=CARTESIAN_POINT('Ctrl Pts',(-20.7394430352779,19.8891498597325,
-8.75237641128897));
#107092=CARTESIAN_POINT('Ctrl Pts',(-20.7148521353619,19.9618707314692,
-8.75700198986289));
#107093=CARTESIAN_POINT('Ctrl Pts',(-20.6863354068359,20.0331529809764,
-8.76162756843682));
#107094=CARTESIAN_POINT('Ctrl Pts',(-20.6540955877885,20.1025839465552,
-8.76625314701075));
#107095=CARTESIAN_POINT('Ctrl Pts',(-20.6367568977556,20.1399241682573,
-8.76874079971745));
#107096=CARTESIAN_POINT('Ctrl Pts',(-20.6183421527917,20.1767293760292,
-8.77122845242414));
#107097=CARTESIAN_POINT('Ctrl Pts',(-20.5988881380091,20.2129387370059,
-8.77371610513084));
#107098=CARTESIAN_POINT('Ctrl Pts',(-20.5645713376049,20.2768118977537,
-8.77810431406173));
#107099=CARTESIAN_POINT('Ctrl Pts',(-20.5269022333032,20.3390446523177,
-8.78249252299262));
#107100=CARTESIAN_POINT('Ctrl Pts',(-20.4860618340585,20.399262735945,-8.78688073192352));
#107101=CARTESIAN_POINT('Ctrl Pts',(-20.4452820487377,20.459391445952,-8.79126242802478));
#107102=CARTESIAN_POINT('Ctrl Pts',(-20.4013405804888,20.5175110248669,
-8.79564412412605));
#107103=CARTESIAN_POINT('Ctrl Pts',(-20.3544642120284,20.5732719029384,
-8.80002582022731));
#107104=CARTESIAN_POINT('Ctrl Pts',(-20.3076429270315,20.6289672575405,
-8.80440236748695));
#107105=CARTESIAN_POINT('Ctrl Pts',(-20.2578939016355,20.6823090498171,
-8.80877891474658));
#107106=CARTESIAN_POINT('Ctrl Pts',(-20.2054860875607,20.732978217359,-8.81315546200621));
#107107=CARTESIAN_POINT('Ctrl Pts',(-20.1531115097599,20.7836152512513,
-8.81752923372318));
#107108=CARTESIAN_POINT('Ctrl Pts',(-20.0980818347941,20.8315826889225,
-8.82190300544015));
#107109=CARTESIAN_POINT('Ctrl Pts',(-20.0407040448455,20.8765970518659,
-8.82627677715712));
#107110=CARTESIAN_POINT('Ctrl Pts',(-19.9833437151512,20.9215977167874,
-8.83064921792067));
#107111=CARTESIAN_POINT('Ctrl Pts',(-19.9236370683482,20.9636467934742,
-8.83502165868421));
#107112=CARTESIAN_POINT('Ctrl Pts',(-19.8619241653176,21.0025010681807,
-8.83939409944776));
#107113=CARTESIAN_POINT('Ctrl Pts',(-19.8002096842813,21.0413563363953,
-8.8437666520151));
#107114=CARTESIAN_POINT('Ctrl Pts',(-19.7364892544409,21.0770163851234,
-8.84813920458243));
#107115=CARTESIAN_POINT('Ctrl Pts',(-19.6711304798876,21.1092822402545,
-8.85251175714977));
#107116=CARTESIAN_POINT('Ctrl Pts',(-19.6057038735327,21.1415815821071,
-8.85688884771709));
#107117=CARTESIAN_POINT('Ctrl Pts',(-19.5386359610959,21.1704794832197,
-8.86126593828441));
#107118=CARTESIAN_POINT('Ctrl Pts',(-19.4703166749626,21.1958241116462,
-8.86564302885173));
#107119=CARTESIAN_POINT('Ctrl Pts',(-19.4019600771315,21.2211825817149,
-8.87002250991067));
#107120=CARTESIAN_POINT('Ctrl Pts',(-19.3323512055658,21.2429837711606,
-8.87440199096961));
#107121=CARTESIAN_POINT('Ctrl Pts',(-19.2618949953294,21.2611258190429,
-8.87878147202854));
#107122=CARTESIAN_POINT('Ctrl Pts',(-19.1913139019334,21.2793000235832,
-8.88316871568826));
#107123=CARTESIAN_POINT('Ctrl Pts',(-19.1198829437791,21.2938020386136,
-8.88755595934798));
#107124=CARTESIAN_POINT('Ctrl Pts',(-19.0480164983111,21.3045812950035,
-8.89194320300769));
#107125=CARTESIAN_POINT('Ctrl Pts',(-18.9991542404263,21.311910150662,-8.89492610594255));
#107126=CARTESIAN_POINT('Ctrl Pts',(-18.9500908178376,21.3175191746182,
-8.89790900887741));
#107127=CARTESIAN_POINT('Ctrl Pts',(-18.9009566611241,21.3214062341896,
-8.90089191181226));
#107128=CARTESIAN_POINT('Ctrl Pts',(-18.8286744078927,21.3271245662635,
-8.90528012074316));
#107129=CARTESIAN_POINT('Ctrl Pts',(-18.7559569381438,21.3291362205188,
-8.90966832967406));
#107130=CARTESIAN_POINT('Ctrl Pts',(-18.6832169260197,21.3273908144284,
-8.91405653860496));
#107131=CARTESIAN_POINT('Ctrl Pts',(-18.6105848721342,21.3256479988102,
-8.91843823470623));
#107132=CARTESIAN_POINT('Ctrl Pts',(-18.5379308205422,21.3201592036426,
-8.92281993080749));
#107133=CARTESIAN_POINT('Ctrl Pts',(-18.4656714572674,21.3109259018249,
-8.92720162690876));
#107134=CARTESIAN_POINT('Ctrl Pts',(-18.393497004495,21.3017034498716,-8.9315781741684));
#107135=CARTESIAN_POINT('Ctrl Pts',(-18.3217167948299,21.2887452929197,
-8.93595472142804));
#107136=CARTESIAN_POINT('Ctrl Pts',(-18.2507446877308,21.2721048743729,
-8.94033126868768));
#107137=CARTESIAN_POINT('Ctrl Pts',(-18.1798175901105,21.2554750089376,
-8.94470504040465));
#107138=CARTESIAN_POINT('Ctrl Pts',(-18.1096980467019,21.2351676251632,
-8.94907881212163));
#107139=CARTESIAN_POINT('Ctrl Pts',(-18.0407905817005,21.2112874049448,
-8.9534525838386));
#107140=CARTESIAN_POINT('Ctrl Pts',(-17.9719040854722,21.1874144515577,
-8.95782502460215));
#107141=CARTESIAN_POINT('Ctrl Pts',(-17.9042293909009,21.1599709780648,
-8.96219746536571));
#107142=CARTESIAN_POINT('Ctrl Pts',(-17.8381550707622,21.1291112748636,
-8.96656990612926));
#107143=CARTESIAN_POINT('Ctrl Pts',(-17.772079061096,21.0982507825765,-8.9709424586966));
#107144=CARTESIAN_POINT('Ctrl Pts',(-17.7076039433216,21.0639740930875,
-8.97531501126394));
#107145=CARTESIAN_POINT('Ctrl Pts',(-17.6450960003,21.0264826023505,-8.97968756383129));
#107146=CARTESIAN_POINT('Ctrl Pts',(-17.5825231841774,20.9889522015303,
-8.98406465439861));
#107147=CARTESIAN_POINT('Ctrl Pts',(-17.5219220335752,20.9482005866783,
-8.98844174496594));
#107148=CARTESIAN_POINT('Ctrl Pts',(-17.4636312781367,20.9044734454698,
-8.99281883553327));
#107149=CARTESIAN_POINT('Ctrl Pts',(-17.4053086879533,20.8607224232466,
-8.99719831659221));
#107150=CARTESIAN_POINT('Ctrl Pts',(-17.3492993758006,20.8139929484573,
-9.00157779765115));
#107151=CARTESIAN_POINT('Ctrl Pts',(-17.2959081742797,20.7645703720129,
-9.0059572787101));
#107152=CARTESIAN_POINT('Ctrl Pts',(-17.2424223372125,20.7150601943836,
-9.01034452236982));
#107153=CARTESIAN_POINT('Ctrl Pts',(-17.1915642147119,20.6628477284534,
-9.01473176602953));
#107154=CARTESIAN_POINT('Ctrl Pts',(-17.1436006220655,20.6082540279654,
-9.01911900968925));
#107155=CARTESIAN_POINT('Ctrl Pts',(-17.1109900008267,20.57113557227,-9.02210191262407));
#107156=CARTESIAN_POINT('Ctrl Pts',(-17.0797165992414,20.5329170566123,
-9.02508481555889));
#107157=CARTESIAN_POINT('Ctrl Pts',(-17.0498528101568,20.4937069980877,
-9.0280677184937));
#107158=CARTESIAN_POINT('Ctrl Pts',(-17.0059195850955,20.4360242867296,
-9.0324559274246));
#107159=CARTESIAN_POINT('Ctrl Pts',(-16.9648675150388,20.3759692727541,
-9.0368441363555));
#107160=CARTESIAN_POINT('Ctrl Pts',(-16.9269623364049,20.3138616787018,
-9.0412323452864));
#107161=CARTESIAN_POINT('Ctrl Pts',(-16.889113415341,20.2518462626167,-9.04561404138767));
#107162=CARTESIAN_POINT('Ctrl Pts',(-16.8544023633226,20.1877847222597,
-9.04999573748894));
#107163=CARTESIAN_POINT('Ctrl Pts',(-16.8230534861161,20.1220282218872,
-9.05437743359021));
#107164=CARTESIAN_POINT('Ctrl Pts',(-16.7917414463352,20.0563489906357,
-9.05875398084985));
#107165=CARTESIAN_POINT('Ctrl Pts',(-16.7637839395866,19.9889791891847,
-9.06313052810949));
#107166=CARTESIAN_POINT('Ctrl Pts',(-16.7393600427009,19.9202957357448,
-9.06750707536913));
#107167=CARTESIAN_POINT('Ctrl Pts',(-16.7149516350957,19.851655840353,-9.07188084708611));
#107168=CARTESIAN_POINT('Ctrl Pts',(-16.694072552212,19.7817043993275,-9.07625461880308));
#107169=CARTESIAN_POINT('Ctrl Pts',(-16.6768537344171,19.7108382158241,
-9.08062839052006));
#107170=CARTESIAN_POINT('Ctrl Pts',(-16.6596401563662,19.6399935971384,
-9.08500083128361));
#107171=CARTESIAN_POINT('Ctrl Pts',(-16.6460847459306,19.5682352570613,
-9.08937327204717));
#107172=CARTESIAN_POINT('Ctrl Pts',(-16.6362680963764,19.4959734382704,
-9.09374571281072));
#107173=CARTESIAN_POINT('Ctrl Pts',(-16.6264511958094,19.4237097717368,
-9.09811826537807));
#107174=CARTESIAN_POINT('Ctrl Pts',(-16.620373308882,19.3509430791855,-9.10249081794542));
#107175=CARTESIAN_POINT('Ctrl Pts',(-16.6180633554341,19.2780903583472,
-9.10686337051276));
#107176=CARTESIAN_POINT('Ctrl Pts',(-16.6157510046294,19.2051620282073,
-9.11124046108009));
#107177=CARTESIAN_POINT('Ctrl Pts',(-16.6172144102078,19.1321479746869,
-9.11561755164742));
#107178=CARTESIAN_POINT('Ctrl Pts',(-16.6224303356468,19.0594660018898,
-9.11999464221475));
#107179=CARTESIAN_POINT('Ctrl Pts',(-16.6276491096962,18.9867443347699,
-9.12437412327369));
#107180=CARTESIAN_POINT('Ctrl Pts',(-16.6366244245267,18.9143555885064,
-9.12875360433264));
#107181=CARTESIAN_POINT('Ctrl Pts',(-16.6492813452852,18.8427105341121,
-9.13313308539158));
#107182=CARTESIAN_POINT('Ctrl Pts',(-16.6619607003507,18.7709384893398,
-9.1375203290513));
#107183=CARTESIAN_POINT('Ctrl Pts',(-16.6783345842871,18.6999132392689,
-9.14190757271103));
#107184=CARTESIAN_POINT('Ctrl Pts',(-16.6982774637592,18.6300329136335,
-9.14629481637075));
#107185=CARTESIAN_POINT('Ctrl Pts',(-16.7118367001087,18.582521025854,-9.14927771930555));
#107186=CARTESIAN_POINT('Ctrl Pts',(-16.7270447244344,18.5355380865901,
-9.15226062224035));
#107187=CARTESIAN_POINT('Ctrl Pts',(-16.7438494759072,18.4892037050155,
-9.15524352517515));
#107188=CARTESIAN_POINT('Ctrl Pts',(-16.7685712862063,18.4210402577036,
-9.15963173410604));
#107189=CARTESIAN_POINT('Ctrl Pts',(-16.79684734214,18.3540153233854,-9.16401994303694));
#107190=CARTESIAN_POINT('Ctrl Pts',(-16.8285526457322,18.2885254040822,
-9.16840815196783));
#107191=CARTESIAN_POINT('Ctrl Pts',(-16.860210893397,18.2231326826776,-9.1727898480691));
#107192=CARTESIAN_POINT('Ctrl Pts',(-16.8952880767682,18.1592708843012,
-9.17717154417036));
#107193=CARTESIAN_POINT('Ctrl Pts',(-16.9336103347363,18.097318693157,-9.18155324027162));
#107194=CARTESIAN_POINT('Ctrl Pts',(-16.9718875610014,18.0354393007677,
-9.18592978753126));
#107195=CARTESIAN_POINT('Ctrl Pts',(-17.0134020343725,17.9754654662074,
-9.1903063347909));
#107196=CARTESIAN_POINT('Ctrl Pts',(-17.0579337571748,17.9177517834298,
-9.19468288205053));
#107197=CARTESIAN_POINT('Ctrl Pts',(-17.1024372386058,17.8600747018311,
-9.1990566537675));
#107198=CARTESIAN_POINT('Ctrl Pts',(-17.1499538788908,17.8046553090193,
-9.20343042548448));
#107199=CARTESIAN_POINT('Ctrl Pts',(-17.2002209049087,17.7518184871439,
-9.20780419720145));
#107200=CARTESIAN_POINT('Ctrl Pts',(-17.2504726345018,17.6989977436909,
-9.212176637965));
#107201=CARTESIAN_POINT('Ctrl Pts',(-17.3034727559329,17.6487583602256,
-9.21654907872854));
#107202=CARTESIAN_POINT('Ctrl Pts',(-17.358919943639,17.6013901595112,-9.22092151949209));
#107203=CARTESIAN_POINT('Ctrl Pts',(-17.4143685491359,17.5540207475868,
-9.22529407205944));
#107204=CARTESIAN_POINT('Ctrl Pts',(-17.4722639770751,17.5095229759788,
-9.22966662462678));
#107205=CARTESIAN_POINT('Ctrl Pts',(-17.5322712521174,17.4681468746585,
-9.23403917719411));
#107206=CARTESIAN_POINT('Ctrl Pts',(-17.5923408049732,17.4267278316597,
-9.23841626776144));
#107207=CARTESIAN_POINT('Ctrl Pts',(-17.6545261829432,17.3884372018126,
-9.24279335832876));
#107208=CARTESIAN_POINT('Ctrl Pts',(-17.7184635014061,17.3534815963163,
-9.24717044889609));
#107209=CARTESIAN_POINT('Ctrl Pts',(-17.7824357384117,17.3185069002664,
-9.25154992995503));
#107210=CARTESIAN_POINT('Ctrl Pts',(-17.8481613859391,17.2868710642732,
-9.25592941101397));
#107211=CARTESIAN_POINT('Ctrl Pts',(-17.9152544897581,17.2587334225422,
-9.26030889207291));
#107212=CARTESIAN_POINT('Ctrl Pts',(-17.9824665156532,17.2305459070301,
-9.26469613573263));
#107213=CARTESIAN_POINT('Ctrl Pts',(-18.0510503837927,17.2058691314343,
-9.26908337939234));
#107214=CARTESIAN_POINT('Ctrl Pts',(-18.1206033812623,17.1848130421599,
-9.27347062305206));
#107215=CARTESIAN_POINT('Ctrl Pts',(-18.167892717431,17.1704969304132,-9.2764535259869));
#107216=CARTESIAN_POINT('Ctrl Pts',(-18.2156297492657,17.1578534982273,
-9.27943642892174));
#107217=CARTESIAN_POINT('Ctrl Pts',(-18.2636857248405,17.1469037128609,
-9.28241933185657));
#107218=CARTESIAN_POINT('Ctrl Pts',(-18.3343818439592,17.1307952618032,
-9.28680754078747));
#107219=CARTESIAN_POINT('Ctrl Pts',(-18.4060444995741,17.1182916243426,
-9.29119574971837));
#107220=CARTESIAN_POINT('Ctrl Pts',(-18.4782726371995,17.1095023159863,
-9.29558395864926));
#107221=CARTESIAN_POINT('Ctrl Pts',(-18.5503935762931,17.1007260524208,
-9.29996565475053));
#107222=CARTESIAN_POINT('Ctrl Pts',(-18.6230778564464,17.0956532323251,
-9.3043473508518));
#107223=CARTESIAN_POINT('Ctrl Pts',(-18.6959129564509,17.0943426405973,
-9.30872904695306));
#107224=CARTESIAN_POINT('Ctrl Pts',(-18.7686624694164,17.0930335889191,
-9.3131055942127));
#107225=CARTESIAN_POINT('Ctrl Pts',(-18.8415619702681,17.0954779920626,
-9.31748214147234));
#107226=CARTESIAN_POINT('Ctrl Pts',(-18.9141942210378,17.1016828017805,
-9.32185868873198));
#107227=CARTESIAN_POINT('Ctrl Pts',(-18.9867804094896,17.1078836764983,
-9.32623246044896));
#107228=CARTESIAN_POINT('Ctrl Pts',(-19.0590992046971,17.1178401850896,
-9.33060623216593));
#107229=CARTESIAN_POINT('Ctrl Pts',(-19.13073519808,17.1315072294897,-9.33498000388291));
#107230=CARTESIAN_POINT('Ctrl Pts',(-19.2023493923895,17.1451701149624,
-9.33935244464646));
#107231=CARTESIAN_POINT('Ctrl Pts',(-19.2732807238328,17.1625412042304,
-9.34372488541001));
#107232=CARTESIAN_POINT('Ctrl Pts',(-19.3431223955196,17.1835240057459,
-9.34809732617357));
#107233=CARTESIAN_POINT('Ctrl Pts',(-19.4129658530657,17.204507343794,-9.35246987874091));
#107234=CARTESIAN_POINT('Ctrl Pts',(-19.4817191341329,17.2291024367364,
-9.35684243130826));
#107235=CARTESIAN_POINT('Ctrl Pts',(-19.5489906872857,17.2571629598051,
-9.36121498387561));
#107236=CARTESIAN_POINT('Ctrl Pts',(-19.6163320573938,17.285252605143,-9.36559207444294));
#107237=CARTESIAN_POINT('Ctrl Pts',(-19.6821881831278,17.3168146752694,
-9.36996916501026));
#107238=CARTESIAN_POINT('Ctrl Pts',(-19.7461883733225,17.3516550355271,
-9.37434625557759));
#107239=CARTESIAN_POINT('Ctrl Pts',(-19.8102235163965,17.3865144233986,
-9.37872573663653));
#107240=CARTESIAN_POINT('Ctrl Pts',(-19.8724002944083,17.424655413658,-9.38310521769548));
#107241=CARTESIAN_POINT('Ctrl Pts',(-19.9323758228016,17.4658397244595,
-9.38748469875442));
#107242=CARTESIAN_POINT('Ctrl Pts',(-19.9924576574163,17.5070970341754,
-9.39187194241414));
#107243=CARTESIAN_POINT('Ctrl Pts',(-20.050330067536,17.5514081430505,-9.39625918607386));
#107244=CARTESIAN_POINT('Ctrl Pts',(-20.1056826247707,17.598493945158,-9.40064642973358));
#107245=CARTESIAN_POINT('Ctrl Pts',(-20.1433170299306,17.630507753414,-9.40362933266839));
#107246=CARTESIAN_POINT('Ctrl Pts',(-20.1797873054598,17.663803392597,-9.4066122356032));
#107247=CARTESIAN_POINT('Ctrl Pts',(-20.2150061302365,17.6982839518925,
-9.40959513853801));
#107248=CARTESIAN_POINT('Ctrl Pts',(-20.2660736595565,17.7482809913723,
-9.41392036756108));
#107249=CARTESIAN_POINT('Ctrl Pts',(-20.3147200093818,17.8009782881339,
-9.41824559658415));
#107250=CARTESIAN_POINT('Ctrl Pts',(-20.3606400168152,17.8561083970681,
-9.42257082560722));
#107251=CARTESIAN_POINT('Ctrl Pts',(-20.4064831242367,17.9111461822795,
-9.42688881137877));
#107252=CARTESIAN_POINT('Ctrl Pts',(-20.4496086380981,17.9686083126782,
-9.43120679715031));
#107253=CARTESIAN_POINT('Ctrl Pts',(-20.489747535905,18.0281899602372,-9.43552478292186));
#107254=CARTESIAN_POINT('Ctrl Pts',(-20.5298476914497,18.087714099296,-9.43983860095224));
#107255=CARTESIAN_POINT('Ctrl Pts',(-20.5669666687477,18.1493532900628,
-9.44415241898263));
#107256=CARTESIAN_POINT('Ctrl Pts',(-20.6008760498721,18.2127701595255,
-9.44846623701301));
#107257=CARTESIAN_POINT('Ctrl Pts',(-20.6347648510145,18.276148540582,-9.45277743693906));
#107258=CARTESIAN_POINT('Ctrl Pts',(-20.6654476851552,18.3413020229497,
-9.45708863686511));
#107259=CARTESIAN_POINT('Ctrl Pts',(-20.692740781525,18.4078664178416,-9.46139983679116));
#107260=CARTESIAN_POINT('Ctrl Pts',(-20.7031862293494,18.433341538157,-9.46304979300271));
#107261=CARTESIAN_POINT('Ctrl Pts',(-20.7131356639248,18.4590230623861,
-9.46469974921426));
#107262=CARTESIAN_POINT('Ctrl Pts',(-20.7225806137986,18.4848897174502,
-9.46634970542581));
#107263=CARTESIAN_POINT('',(-20.8509991049198,19.2129467328109,-8.4890562790225));
#107264=CARTESIAN_POINT('Ctrl Pts',(-20.7225807588464,18.4848901146894,
-9.24346988827878));
#107265=CARTESIAN_POINT('Ctrl Pts',(-20.6903083395894,18.39650636827,-9.23734843558896));
#107266=CARTESIAN_POINT('Ctrl Pts',(-20.6521496472009,18.3102912124771,
-9.23135300036806));
#107267=CARTESIAN_POINT('Ctrl Pts',(-20.5973016866332,18.2058341370534,
-9.2240858578963));
#107268=CARTESIAN_POINT('Ctrl Pts',(-20.5859225848332,18.1850202735708,
-9.22263722284196));
#107269=CARTESIAN_POINT('Ctrl Pts',(-20.5694165868721,18.1559983874074,
-9.2206157129183));
#107270=CARTESIAN_POINT('Ctrl Pts',(-20.5645798963423,18.1476281469331,
-9.22003249182282));
#107271=CARTESIAN_POINT('Ctrl Pts',(-20.5566541761581,18.1341264602102,
-9.21909131991471));
#107272=CARTESIAN_POINT('Ctrl Pts',(-20.5536004477713,18.1289745482744,
-9.21873209594647));
#107273=CARTESIAN_POINT('Ctrl Pts',(-20.5471836479079,18.1182528241218,
-9.217984278638));
#107274=CARTESIAN_POINT('Ctrl Pts',(-20.5438166747774,18.1126854109202,
-9.21759583267081));
#107275=CARTESIAN_POINT('Ctrl Pts',(-20.5357844895098,18.0995411280695,
-9.21667837924833));
#107276=CARTESIAN_POINT('Ctrl Pts',(-20.5310970461766,18.0919779354556,
-9.21615019438572));
#107277=CARTESIAN_POINT('Ctrl Pts',(-20.5153276832105,18.0668887096903,
-9.2143969132788));
#107278=CARTESIAN_POINT('Ctrl Pts',(-20.5040357536673,18.0494956154335,
-9.21317959276562));
#107279=CARTESIAN_POINT('Ctrl Pts',(-20.4423940085405,17.9575352427292,
-9.20672866183974));
#107280=CARTESIAN_POINT('Ctrl Pts',(-20.3875818629946,17.8860646473677,
-9.20166799572178));
#107281=CARTESIAN_POINT('Ctrl Pts',(-20.239237271279,17.7162386259572,-9.18923109939529));
#107282=CARTESIAN_POINT('Ctrl Pts',(-20.1405044242798,17.6229842972969,
-9.18201885997539));
#107283=CARTESIAN_POINT('Ctrl Pts',(-19.9740224059233,17.4935257233293,
-9.17034301708339));
#107284=CARTESIAN_POINT('Ctrl Pts',(-19.9120806441693,17.4504611918285,
-9.16608238927342));
#107285=CARTESIAN_POINT('Ctrl Pts',(-19.8399125093472,17.4058028978743,
-9.16105250608856));
#107286=CARTESIAN_POINT('Ctrl Pts',(-19.8318095060137,17.400863724253,-9.16048684628342));
#107287=CARTESIAN_POINT('Ctrl Pts',(-19.8197475229313,17.3936221394976,
-9.15964305507023));
#107288=CARTESIAN_POINT('Ctrl Pts',(-19.8158137093209,17.3912777495406,
-9.1593675912986));
#107289=CARTESIAN_POINT('Ctrl Pts',(-19.8087982558611,17.3871276178277,
-9.15887579078604));
#107290=CARTESIAN_POINT('Ctrl Pts',(-19.8057196225779,17.3853168928855,
-9.15865978255638));
#107291=CARTESIAN_POINT('Ctrl Pts',(-19.7990875252467,17.3814387235023,
-9.15819402960866));
#107292=CARTESIAN_POINT('Ctrl Pts',(-19.7955326690794,17.3793738665576,
-9.157944128941));
#107293=CARTESIAN_POINT('Ctrl Pts',(-19.7856957203983,17.3736982789767,
-9.15725195721474));
#107294=CARTESIAN_POINT('Ctrl Pts',(-19.7794011390049,17.3701094661957,
-9.15680831255862));
#107295=CARTESIAN_POINT('Ctrl Pts',(-19.7446856398884,17.3505521283599,
-9.15435807751532));
#107296=CARTESIAN_POINT('Ctrl Pts',(-19.7159188643973,17.3352103479093,
-9.15231500282216));
#107297=CARTESIAN_POINT('Ctrl Pts',(-19.5415662171688,17.2473348280452,
-9.13990762731865));
#107298=CARTESIAN_POINT('Ctrl Pts',(-19.3883729642573,17.1911138485735,
-9.12895444031794));
#107299=CARTESIAN_POINT('Ctrl Pts',(-19.1167166811949,17.1256085732853,
-9.11070156650593));
#107300=CARTESIAN_POINT('Ctrl Pts',(-19.0010936888834,17.1076697300265,
-9.10326200789545));
#107301=CARTESIAN_POINT('Ctrl Pts',(-18.8703108408879,17.0983446725026,
-9.09525614356276));
#107302=CARTESIAN_POINT('Ctrl Pts',(-18.8560477444649,17.0974727250556,
-9.09438818313206));
#107303=CARTESIAN_POINT('Ctrl Pts',(-18.8333331565297,17.0963148221154,
-9.09301389449998));
#107304=CARTESIAN_POINT('Ctrl Pts',(-18.8248870837847,17.0959349847366,
-9.0925046383631));
#107305=CARTESIAN_POINT('Ctrl Pts',(-18.8099870560799,17.0953543169118,
-9.09160926540666));
#107306=CARTESIAN_POINT('Ctrl Pts',(-18.8035340756784,17.0951323995075,
-9.09122249248421));
#107307=CARTESIAN_POINT('Ctrl Pts',(-18.7901850998829,17.0947344641633,
-9.09042442269024));
#107308=CARTESIAN_POINT('Ctrl Pts',(-18.7832890495817,17.0945626220126,
-9.09001326121201));
#107309=CARTESIAN_POINT('Ctrl Pts',(-18.7655855987095,17.0942080452139,
-9.08896054167088));
#107310=CARTESIAN_POINT('Ctrl Pts',(-18.7547773312555,17.0940743662193,
-9.0883205249654));
#107311=CARTESIAN_POINT('Ctrl Pts',(-18.7096624307513,17.0938619304368,
-9.085659783059));
#107312=CARTESIAN_POINT('Ctrl Pts',(-18.6753563294909,17.0945343046956,
-9.08366258832262));
#107313=CARTESIAN_POINT('Ctrl Pts',(-18.5860257293788,17.0984590033235,
-9.07851830035413));
#107314=CARTESIAN_POINT('Ctrl Pts',(-18.5310841793984,17.1030266456553,
-9.0754106003379));
#107315=CARTESIAN_POINT('Ctrl Pts',(-18.3678444459834,17.123040178458,-9.06626594373675));
#107316=CARTESIAN_POINT('Ctrl Pts',(-18.2604997145706,17.1447365925,-9.06037771571652));
#107317=CARTESIAN_POINT('Ctrl Pts',(-18.1111197350522,17.1871868071586,
-9.05192281864917));
#107318=CARTESIAN_POINT('Ctrl Pts',(-18.0673492586714,17.201180054876,-9.04941075452979));
#107319=CARTESIAN_POINT('Ctrl Pts',(-18.003068890374,17.2240612375143,-9.045626788143));
#107320=CARTESIAN_POINT('Ctrl Pts',(-17.9821876135874,17.2318678619025,
-9.04438233540202));
#107321=CARTESIAN_POINT('Ctrl Pts',(-17.9135808826573,17.2587594368671,
-9.04023136472835));
#107322=CARTESIAN_POINT('Ctrl Pts',(-17.866430766497,17.2792511943401,-9.03727797782522));
#107323=CARTESIAN_POINT('Ctrl Pts',(-17.8129718908838,17.3048367666467,
-9.03376035406435));
#107324=CARTESIAN_POINT('Ctrl Pts',(-17.8058857238463,17.3082769681307,
-9.03329057397738));
#107325=CARTESIAN_POINT('Ctrl Pts',(-17.7946183282661,17.3138249951052,
-9.03253773336924));
#107326=CARTESIAN_POINT('Ctrl Pts',(-17.7904245305458,17.3159073223538,
-9.03225621795564));
#107327=CARTESIAN_POINT('Ctrl Pts',(-17.7830248264716,17.319612115509,-9.03175713356468));
#107328=CARTESIAN_POINT('Ctrl Pts',(-17.7798160995386,17.3212288513649,
-9.03153992450984));
#107329=CARTESIAN_POINT('Ctrl Pts',(-17.773041017024,17.324664171307,-9.03107959958146));
#107330=CARTESIAN_POINT('Ctrl Pts',(-17.769475755008,17.3264846761617,-9.03083636882649));
#107331=CARTESIAN_POINT('Ctrl Pts',(-17.759905226379,17.3314058816175,-9.03018081430051));
#107332=CARTESIAN_POINT('Ctrl Pts',(-17.7539096684074,17.3345252154846,
-9.02976734263338));
#107333=CARTESIAN_POINT('Ctrl Pts',(-17.724704962782,17.3498978165027,-9.02774000926112));
#107334=CARTESIAN_POINT('Ctrl Pts',(-17.7017112284554,17.3625526636707,
-9.02610270299731));
#107335=CARTESIAN_POINT('Ctrl Pts',(-17.6365230815829,17.4000252945157,
-9.02135462931007));
#107336=CARTESIAN_POINT('Ctrl Pts',(-17.5949477248333,17.4258825662844,
-9.01819628861483));
#107337=CARTESIAN_POINT('Ctrl Pts',(-17.4740574198348,17.5070121729297,
-9.00869584960283));
#107338=CARTESIAN_POINT('Ctrl Pts',(-17.3975893964271,17.5663005383351,
-9.00226695202653));
#107339=CARTESIAN_POINT('Ctrl Pts',(-17.2201677022836,17.7244313396584,
-8.98663144364373));
#107340=CARTESIAN_POINT('Ctrl Pts',(-17.1245173602814,17.8285552124252,
-8.97756391735156));
#107341=CARTESIAN_POINT('Ctrl Pts',(-17.0313565068578,17.9528672074506,
-8.96807857658354));
#107342=CARTESIAN_POINT('Ctrl Pts',(-17.0229070615236,17.9643829938517,
-8.96721102492995));
#107343=CARTESIAN_POINT('Ctrl Pts',(-17.0096436064228,17.9828487581173,
-8.96583725915923));
#107344=CARTESIAN_POINT('Ctrl Pts',(-17.0047536795196,17.9897434293522,
-8.96532812057188));
#107345=CARTESIAN_POINT('Ctrl Pts',(-16.9962016695629,18.0019558950485,
-8.96443288433582));
#107346=CARTESIAN_POINT('Ctrl Pts',(-16.9925223996357,18.0072614678221,
-8.96404613121473));
#107347=CARTESIAN_POINT('Ctrl Pts',(-16.9849620336064,18.0182708662349,
-8.96324803527219));
#107348=CARTESIAN_POINT('Ctrl Pts',(-16.9810844276534,18.0239770042768,
-8.96283682817445));
#107349=CARTESIAN_POINT('Ctrl Pts',(-16.9712013946726,18.0386745400552,
-8.96178385308575));
#107350=CARTESIAN_POINT('Ctrl Pts',(-16.9652367856299,18.0476932455129,
-8.96114362792164));
#107351=CARTESIAN_POINT('Ctrl Pts',(-16.9406198414327,18.0855420216681,
-8.95848085909162));
#107352=CARTESIAN_POINT('Ctrl Pts',(-16.9226006072697,18.1147789952353,
-8.95648189167311));
#107353=CARTESIAN_POINT('Ctrl Pts',(-16.8775016624623,18.1921048423589,
-8.95133200470345));
#107354=CARTESIAN_POINT('Ctrl Pts',(-16.8515762352676,18.2408377264412,
-8.94822059091668));
#107355=CARTESIAN_POINT('Ctrl Pts',(-16.7800137119302,18.389053436859,-8.93906945594282));
#107356=CARTESIAN_POINT('Ctrl Pts',(-16.7401520658335,18.4911181633063,
-8.93317844158517));
#107357=CARTESIAN_POINT('Ctrl Pts',(-16.6935664703212,18.6445100468694,
-8.92445019024973));
#107358=CARTESIAN_POINT('Ctrl Pts',(-16.6805367772416,18.6937299550284,
-8.92166567303186));
#107359=CARTESIAN_POINT('Ctrl Pts',(-16.6658192487566,18.7587115674047,
-8.917958809007));
#107360=CARTESIAN_POINT('Ctrl Pts',(-16.6625156761329,18.7740914001609,
-8.91707922224968));
#107361=CARTESIAN_POINT('Ctrl Pts',(-16.6488821027157,18.8411966359645,
-8.91322628594086));
#107362=CARTESIAN_POINT('Ctrl Pts',(-16.6403167641891,18.8932568753744,
-8.91019833674597));
#107363=CARTESIAN_POINT('Ctrl Pts',(-16.6326149766072,18.9542013648139,
-8.90655274116614));
#107364=CARTESIAN_POINT('Ctrl Pts',(-16.6315783129375,18.9628315098977,
-8.90603415520237));
#107365=CARTESIAN_POINT('Ctrl Pts',(-16.6300882631837,18.9759160808096,
-8.90524402113409));
#107366=CARTESIAN_POINT('Ctrl Pts',(-16.6295957989255,18.9803660843912,
-8.90497462085352));
#107367=CARTESIAN_POINT('Ctrl Pts',(-16.6287367224929,18.9883607592236,
-8.90448935550362));
#107368=CARTESIAN_POINT('Ctrl Pts',(-16.6283649411118,18.9919048206068,
-8.90427378448645));
#107369=CARTESIAN_POINT('Ctrl Pts',(-16.6275760431054,18.99961262089,-8.90380395693945));
#107370=CARTESIAN_POINT('Ctrl Pts',(-16.6271623281248,19.0037766087173,
-8.90354951746798));
#107371=CARTESIAN_POINT('Ctrl Pts',(-16.6260337072066,19.0154888838935,
-8.90283213906703));
#107372=CARTESIAN_POINT('Ctrl Pts',(-16.6253470121312,19.0230397360276,
-8.90236766099264));
#107373=CARTESIAN_POINT('Ctrl Pts',(-16.6214621588587,19.0684612666666,
-8.89956235031418));
#107374=CARTESIAN_POINT('Ctrl Pts',(-16.6192439489004,19.1064062636917,
-8.89717176310606));
#107375=CARTESIAN_POINT('Ctrl Pts',(-16.6152879466501,19.2320690459693,
-8.88914355983114));
#107376=CARTESIAN_POINT('Ctrl Pts',(-16.6179805449662,19.3198319840568,
-8.88336095675132));
#107377=CARTESIAN_POINT('Ctrl Pts',(-16.6422709203489,19.5808395850592,
-8.86604060451694));
#107378=CARTESIAN_POINT('Ctrl Pts',(-16.6798383616897,19.7518834242279,
-8.85459345794534));
#107379=CARTESIAN_POINT('Ctrl Pts',(-16.7456645980709,19.9381474156945,
-8.84243278823315));
#107380=CARTESIAN_POINT('Ctrl Pts',(-16.753705457454,19.9597687396893,-8.84102462834996));
#107381=CARTESIAN_POINT('Ctrl Pts',(-16.7655760968599,19.990158328726,-8.83904959752108));
#107382=CARTESIAN_POINT('Ctrl Pts',(-16.7691141662067,19.9990380882435,
-8.83847300682397));
#107383=CARTESIAN_POINT('Ctrl Pts',(-16.7749591998491,20.0134236865229,
-8.8375396492632));
#107384=CARTESIAN_POINT('Ctrl Pts',(-16.7772294943446,20.0189441928006,
-8.83718165019393));
#107385=CARTESIAN_POINT('Ctrl Pts',(-16.7820294167997,20.0304768979414,
-8.83643411163075));
#107386=CARTESIAN_POINT('Ctrl Pts',(-16.7845635463761,20.036487164461,-8.83604472949029));
#107387=CARTESIAN_POINT('Ctrl Pts',(-16.790656012413,20.0507523135977,-8.83512096642121));
#107388=CARTESIAN_POINT('Ctrl Pts',(-16.794239246073,20.058996476174,-8.83458743957967));
#107389=CARTESIAN_POINT('Ctrl Pts',(-16.806477042741,20.0866692351083,-8.83279751320582));
#107390=CARTESIAN_POINT('Ctrl Pts',(-16.815372026829,20.105990563738,-8.83154934939907));
#107391=CARTESIAN_POINT('Ctrl Pts',(-16.8912560756496,20.2644900374526,
-8.82131541919827));
#107392=CARTESIAN_POINT('Ctrl Pts',(-16.9730020083597,20.3960906972459,
-8.81289814565379));
#107393=CARTESIAN_POINT('Ctrl Pts',(-17.1527684397966,20.6252498445392,
-8.79708144219461));
#107394=CARTESIAN_POINT('Ctrl Pts',(-17.2474050757665,20.7244136970755,
-8.78969581197635));
#107395=CARTESIAN_POINT('Ctrl Pts',(-17.3627251487734,20.823928150583,-8.78076356911416));
#107396=CARTESIAN_POINT('Ctrl Pts',(-17.3746370788697,20.8339800840723,
-8.77984146474872));
#107397=CARTESIAN_POINT('Ctrl Pts',(-17.3911125734593,20.8475743811132,
-8.77856511293135));
#107398=CARTESIAN_POINT('Ctrl Pts',(-17.3955815886669,20.8512312336081,
-8.77821880218579));
#107399=CARTESIAN_POINT('Ctrl Pts',(-17.402711805465,20.857017119495,-8.7776660146463));
#107400=CARTESIAN_POINT('Ctrl Pts',(-17.4053633214568,20.8591581206392,
-8.77746039342052));
#107401=CARTESIAN_POINT('Ctrl Pts',(-17.410854403414,20.8635701046648,-8.77703442534781));
#107402=CARTESIAN_POINT('Ctrl Pts',(-17.4136946459747,20.8658401711196,
-8.77681401328082));
#107403=CARTESIAN_POINT('Ctrl Pts',(-17.4204832662322,20.8712373803497,
-8.77628702455514));
#107404=CARTESIAN_POINT('Ctrl Pts',(-17.4244369713162,20.8743577611866,
-8.77597997029093));
#107405=CARTESIAN_POINT('Ctrl Pts',(-17.4378411345816,20.884859309836,-8.77493862502507));
#107406=CARTESIAN_POINT('Ctrl Pts',(-17.4473429581101,20.8921741238841,
-8.77419986816113));
#107407=CARTESIAN_POINT('Ctrl Pts',(-17.5586199792945,20.9763428973501,
-8.76554655148382));
#107408=CARTESIAN_POINT('Ctrl Pts',(-17.667067384525,21.043921653715,-8.75711299323475));
#107409=CARTESIAN_POINT('Ctrl Pts',(-17.9283045479755,21.1756341474197,
-8.73777924048841));
#107410=CARTESIAN_POINT('Ctrl Pts',(-18.0838999539409,21.2324653363557,
-8.72698402934422));
#107411=CARTESIAN_POINT('Ctrl Pts',(-18.2675081867491,21.276098454808,-8.71536087180296));
#107412=CARTESIAN_POINT('Ctrl Pts',(-18.2905648925023,21.2811718808147,
-8.71391924262907));
#107413=CARTESIAN_POINT('Ctrl Pts',(-18.323158379011,21.2877742407969,-8.71190578414224));
#107414=CARTESIAN_POINT('Ctrl Pts',(-18.3326274726973,21.2896250705507,
-8.71132371824018));
#107415=CARTESIAN_POINT('Ctrl Pts',(-18.3479909601404,21.2925191198023,
-8.71038390884797));
#107416=CARTESIAN_POINT('Ctrl Pts',(-18.3538776263852,21.2936021720859,
-8.71002489936757));
#107417=CARTESIAN_POINT('Ctrl Pts',(-18.3661753534045,21.2958108778802,
-8.70927713734061));
#107418=CARTESIAN_POINT('Ctrl Pts',(-18.3725871795826,21.2969319600285,
-8.70888853388355));
#107419=CARTESIAN_POINT('Ctrl Pts',(-18.3877912319547,21.2995181196459,
-8.70797000841313));
#107420=CARTESIAN_POINT('Ctrl Pts',(-18.3965877860205,21.3009572839462,
-8.70744091433629));
#107421=CARTESIAN_POINT('Ctrl Pts',(-18.4253807082772,21.3054814378798,
-8.70571651322996));
#107422=CARTESIAN_POINT('Ctrl Pts',(-18.4454126279572,21.3083353883952,
-8.70452851777621));
#107423=CARTESIAN_POINT('Ctrl Pts',(-18.4930782464337,21.3144304510945,
-8.70172751204178));
#107424=CARTESIAN_POINT('Ctrl Pts',(-18.520741291133,21.317414911011,-8.7001224606839));
#107425=CARTESIAN_POINT('Ctrl Pts',(-18.7171632174364,21.3346967664227,
-8.68885184275668));
#107426=CARTESIAN_POINT('Ctrl Pts',(-18.8870366382803,21.3292431036846,
-8.67982469425932));
#107427=CARTESIAN_POINT('Ctrl Pts',(-19.1572083200178,21.2878703031383,
-8.66488782810029));
#107428=CARTESIAN_POINT('Ctrl Pts',(-19.2586531281362,21.2645892464582,
-8.65912345852071));
#107429=CARTESIAN_POINT('Ctrl Pts',(-19.3672203720451,21.231102674287,-8.65239239498147));
#107430=CARTESIAN_POINT('Ctrl Pts',(-19.3764579479185,21.2281838367725,
-8.65181508283472));
#107431=CARTESIAN_POINT('Ctrl Pts',(-19.3900688511936,21.223780164267,-8.65095721441388));
#107432=CARTESIAN_POINT('Ctrl Pts',(-19.3944580257278,21.2223442078616,
-8.65067945663196));
#107433=CARTESIAN_POINT('Ctrl Pts',(-19.402237097736,21.2197710088452,-8.65018513623201));
#107434=CARTESIAN_POINT('Ctrl Pts',(-19.4056288494964,21.2186395276747,
-8.64996891512292));
#107435=CARTESIAN_POINT('Ctrl Pts',(-19.4128905138738,21.2161965903029,
-8.64950448804922));
#107436=CARTESIAN_POINT('Ctrl Pts',(-19.4167594426001,21.2148825410882,
-8.64925613549996));
#107437=CARTESIAN_POINT('Ctrl Pts',(-19.427371073762,21.2112440904193,-8.64857250172216));
#107438=CARTESIAN_POINT('Ctrl Pts',(-19.4341057996568,21.2088968274504,
-8.64813590107006));
#107439=CARTESIAN_POINT('Ctrl Pts',(-19.469522545189,21.1963519181368,-8.64582597643536));
#107440=CARTESIAN_POINT('Ctrl Pts',(-19.4979924242387,21.1855710942037,
-8.64392094984173));
#107441=CARTESIAN_POINT('Ctrl Pts',(-19.6765791192122,21.113504567797,-8.63170751631969));
#107442=CARTESIAN_POINT('Ctrl Pts',(-19.819466720913,21.0357575906665,-8.62079152232837));
#107443=CARTESIAN_POINT('Ctrl Pts',(-20.0499071872592,20.8736437336749,
-8.60236926501126));
#107444=CARTESIAN_POINT('Ctrl Pts',(-20.1417396485142,20.7966460337832,
-8.59474165427677));
#107445=CARTESIAN_POINT('Ctrl Pts',(-20.237728804307,20.7012132347215,-8.58647646815566));
#107446=CARTESIAN_POINT('Ctrl Pts',(-20.2487462297809,20.690013077051,-8.58552266149275));
#107447=CARTESIAN_POINT('Ctrl Pts',(-20.2652268072771,20.6728818162581,
-8.58408773358543));
#107448=CARTESIAN_POINT('Ctrl Pts',(-20.270782249834,20.6670406242377,-8.58360259570072));
#107449=CARTESIAN_POINT('Ctrl Pts',(-20.2806777383336,20.6565164254353,
-8.5827358061962));
#107450=CARTESIAN_POINT('Ctrl Pts',(-20.285030195311,20.6518452717336,-8.58235362189488));
#107451=CARTESIAN_POINT('Ctrl Pts',(-20.2942209544187,20.6418916398686,
-8.58154456269921));
#107452=CARTESIAN_POINT('Ctrl Pts',(-20.2990537199674,20.6366041411294,
-8.58111792659856));
#107453=CARTESIAN_POINT('Ctrl Pts',(-20.3088371056724,20.6257904914001,
-8.58025171602067));
#107454=CARTESIAN_POINT('Ctrl Pts',(-20.3137857015481,20.6202626381434,
-8.57981222978447));
#107455=CARTESIAN_POINT('Ctrl Pts',(-20.335574356308,20.5956645210763,-8.57787103507855));
#107456=CARTESIAN_POINT('Ctrl Pts',(-20.3520993621153,20.5763171027709,
-8.57638243280682));
#107457=CARTESIAN_POINT('Ctrl Pts',(-20.4222714019905,20.4910958303987,
-8.56998131244689));
#107458=CARTESIAN_POINT('Ctrl Pts',(-20.4722775266332,20.4223212234805,
-8.56521408864848));
#107459=CARTESIAN_POINT('Ctrl Pts',(-20.5551898596844,20.2925375571772,
-8.5567264422167));
#107460=CARTESIAN_POINT('Ctrl Pts',(-20.5894925766467,20.2325692067203,
-8.55298131127313));
#107461=CARTESIAN_POINT('Ctrl Pts',(-20.6801422932605,20.054410133297,-8.54212544850229));
#107462=CARTESIAN_POINT('Ctrl Pts',(-20.7285327012151,19.932554217635,-8.53503491361746));
#107463=CARTESIAN_POINT('Ctrl Pts',(-20.769799326511,19.7919117142914,-8.52644208282981));
#107464=CARTESIAN_POINT('Ctrl Pts',(-20.7740668387401,19.7767425016399,
-8.52550998776409));
#107465=CARTESIAN_POINT('Ctrl Pts',(-20.7796729208635,19.7559265525559,
-8.52422191267096));
#107466=CARTESIAN_POINT('Ctrl Pts',(-20.7811583219922,19.7503194319977,
-8.52387405870588));
#107467=CARTESIAN_POINT('Ctrl Pts',(-20.7834811070228,19.7414034703812,
-8.52331941663725));
#107468=CARTESIAN_POINT('Ctrl Pts',(-20.7843335776056,19.7380985387925,
-8.52311349442651));
#107469=CARTESIAN_POINT('Ctrl Pts',(-20.7860768721652,19.7312717633836,
-8.52268742707242));
#107470=CARTESIAN_POINT('Ctrl Pts',(-20.7869666217107,19.7277496941576,
-8.52246721905637));
#107471=CARTESIAN_POINT('Ctrl Pts',(-20.7890638354669,19.7193569746191,
-8.52194157923698));
#107472=CARTESIAN_POINT('Ctrl Pts',(-20.7902630516338,19.7144843024198,
-8.52163567625239));
#107473=CARTESIAN_POINT('Ctrl Pts',(-20.7927674041357,19.7041503872006,
-8.52098545266681));
#107474=CARTESIAN_POINT('Ctrl Pts',(-20.7940681571072,19.6986881331292,
-8.52064089399558));
#107475=CARTESIAN_POINT('Ctrl Pts',(-20.7975804762354,19.683674039106,-8.51969155133116));
#107476=CARTESIAN_POINT('Ctrl Pts',(-20.7997474098406,19.6741120380835,
-8.51908444441543));
#107477=CARTESIAN_POINT('Ctrl Pts',(-20.8343835382445,19.5161922354477,
-8.50902056227148));
#107478=CARTESIAN_POINT('Ctrl Pts',(-20.8508585305448,19.3647964103147,
-8.49886440074919));
#107479=CARTESIAN_POINT('Ctrl Pts',(-20.8509990928577,19.2129598060055,
-8.48885791885903));
#107480=CARTESIAN_POINT('Ctrl Pts',(-20.8509991049198,19.2129467328109,
-8.4890562790225));
#107481=CARTESIAN_POINT('Ctrl Pts',(-20.8510652694519,19.1409952794406,
-8.48473008583438));
#107482=CARTESIAN_POINT('Ctrl Pts',(-20.8474590099797,19.0689489014342,
-8.48040389264625));
#107483=CARTESIAN_POINT('Ctrl Pts',(-20.8401779985051,18.9972168420736,
-8.47607769945812));
#107484=CARTESIAN_POINT('Ctrl Pts',(-20.8329019842487,18.9255340149865,
-8.47175447549083));
#107485=CARTESIAN_POINT('Ctrl Pts',(-20.8219562717615,18.8541655692599,
-8.46743125152355));
#107486=CARTESIAN_POINT('Ctrl Pts',(-20.8073905458164,18.7835182524142,
-8.46310802755626));
#107487=CARTESIAN_POINT('Ctrl Pts',(-20.7928276075188,18.712884456337,-8.45878563098502));
#107488=CARTESIAN_POINT('Ctrl Pts',(-20.7746461242502,18.6429720006697,
-8.45446323441377));
#107489=CARTESIAN_POINT('Ctrl Pts',(-20.7529470567908,18.5741783751506,
-8.45014083784253));
#107490=CARTESIAN_POINT('Ctrl Pts',(-20.7434888020108,18.5441924027759,
-8.44825677862629));
#107491=CARTESIAN_POINT('Ctrl Pts',(-20.7333628777044,18.5144188420078,
-8.44637271941005));
#107492=CARTESIAN_POINT('Ctrl Pts',(-20.7225806137986,18.4848897174502,
-8.44448866019381));
#107493=CARTESIAN_POINT('Origin',(-18.734,19.211,0.));
#107494=CARTESIAN_POINT('',(-20.7249099383763,18.4840591618169,-7.64456003119576));
#107495=CARTESIAN_POINT('',(-20.72258060468,18.4848896924774,-7.86510589144174));
#107496=CARTESIAN_POINT('',(-20.7225806137986,18.4848897174502,0.));
#107497=CARTESIAN_POINT('Ctrl Pts',(-20.72258060468,18.4848896924774,-7.86510589144174));
#107498=CARTESIAN_POINT('Ctrl Pts',(-20.7375769998214,18.525959954405,-7.86752226702014));
#107499=CARTESIAN_POINT('Ctrl Pts',(-20.7513004634184,18.5674931846836,
-7.86996742714882));
#107500=CARTESIAN_POINT('Ctrl Pts',(-20.774507307338,18.6457943285263,-7.87462970750348));
#107501=CARTESIAN_POINT('Ctrl Pts',(-20.7843050079669,18.6824392235647,
-7.87683265697601));
#107502=CARTESIAN_POINT('Ctrl Pts',(-20.7948724777023,18.7266952903225,
-7.87953976353451));
#107503=CARTESIAN_POINT('Ctrl Pts',(-20.7965927836893,18.7340750311575,
-7.8799927178299));
#107504=CARTESIAN_POINT('Ctrl Pts',(-20.7992012895929,18.7455430893457,
-7.88069921951285));
#107505=CARTESIAN_POINT('Ctrl Pts',(-20.8001170723227,18.749625157845,-7.88095121241774));
#107506=CARTESIAN_POINT('Ctrl Pts',(-20.8017905253459,18.7571894193622,
-7.88141916099004));
#107507=CARTESIAN_POINT('Ctrl Pts',(-20.8025515052419,18.7606708210759,
-7.88163492431416));
#107508=CARTESIAN_POINT('Ctrl Pts',(-20.8042489792987,18.7685316732664,
-7.88212299081495));
#107509=CARTESIAN_POINT('Ctrl Pts',(-20.8051803635868,18.77291215825,-7.88239558046764));
#107510=CARTESIAN_POINT('Ctrl Pts',(-20.8078797703266,18.7858090387155,
-7.88319986520688));
#107511=CARTESIAN_POINT('Ctrl Pts',(-20.8096091888307,18.7943332931264,
-7.88373368416764));
#107512=CARTESIAN_POINT('Ctrl Pts',(-20.8214936949608,18.8548223153753,
-7.88753628113026));
#107513=CARTESIAN_POINT('Ctrl Pts',(-20.8297477735186,18.9071369988817,
-7.89090069994371));
#107514=CARTESIAN_POINT('Ctrl Pts',(-20.8378088389374,18.9745650814762,
-7.89528838354835));
#107515=CARTESIAN_POINT('Ctrl Pts',(-20.8394281152034,18.9894474376463,
-7.8962600198513));
#107516=CARTESIAN_POINT('Ctrl Pts',(-20.8475637141893,19.0723916912477,
-7.90168909965173));
#107517=CARTESIAN_POINT('Ctrl Pts',(-20.8509374102031,19.1407195013328,
-7.90621171713557));
#107518=CARTESIAN_POINT('Ctrl Pts',(-20.8511442880123,19.3698585923934,
-7.92135267539541));
#107519=CARTESIAN_POINT('Ctrl Pts',(-20.832975226392,19.5301508319367,-7.9318506755467));
#107520=CARTESIAN_POINT('Ctrl Pts',(-20.7914795966215,19.7100311498939,
-7.94322217798434));
#107521=CARTESIAN_POINT('Ctrl Pts',(-20.7857446856256,19.7331093721006,
-7.94467445754255));
#107522=CARTESIAN_POINT('Ctrl Pts',(-20.777130402795,19.7654373703139,-7.94670015645179));
#107523=CARTESIAN_POINT('Ctrl Pts',(-20.7745746989045,19.7747708253192,
-7.94728397926491));
#107524=CARTESIAN_POINT('Ctrl Pts',(-20.7703333351987,19.7898535533649,
-7.94822586104407));
#107525=CARTESIAN_POINT('Ctrl Pts',(-20.7686871311676,19.7956136909892,
-7.9485851969033));
#107526=CARTESIAN_POINT('Ctrl Pts',(-20.7652024820852,19.8076136017481,
-7.94933304408305));
#107527=CARTESIAN_POINT('Ctrl Pts',(-20.7633596814752,19.813852052895,-7.94972140892112));
#107528=CARTESIAN_POINT('Ctrl Pts',(-20.7589304678799,19.8285958452658,
-7.95063830833244));
#107529=CARTESIAN_POINT('Ctrl Pts',(-20.7563191641273,19.8370936271149,
-7.9511660230735));
#107530=CARTESIAN_POINT('Ctrl Pts',(-20.7474528182278,19.8653124503228,
-7.95291610515229));
#107531=CARTESIAN_POINT('Ctrl Pts',(-20.7409620989911,19.8849586128504,
-7.95413073624497));
#107532=CARTESIAN_POINT('Ctrl Pts',(-20.704833847573,19.9891582238327,-7.96055729785824));
#107533=CARTESIAN_POINT('Ctrl Pts',(-20.6701375233483,20.0718660872074,
-7.96559780859476));
#107534=CARTESIAN_POINT('Ctrl Pts',(-20.5703572156766,20.2729144430854,
-7.97797943898009));
#107535=CARTESIAN_POINT('Ctrl Pts',(-20.4990149366166,20.3876861426273,
-7.98515788350393));
#107536=CARTESIAN_POINT('Ctrl Pts',(-20.370854188125,20.5557113840558,-7.99685014611318));
#107537=CARTESIAN_POINT('Ctrl Pts',(-20.3212057374879,20.6139667239307,
-8.00116972646293));
#107538=CARTESIAN_POINT('Ctrl Pts',(-20.2619779463709,20.6762858434198,
-8.00626509881932));
#107539=CARTESIAN_POINT('Ctrl Pts',(-20.2553888181487,20.683126103271,-8.00683122863796));
#107540=CARTESIAN_POINT('Ctrl Pts',(-20.2455537544683,20.6931994579397,
-8.0076755881059));
#107541=CARTESIAN_POINT('Ctrl Pts',(-20.2423428874341,20.6964668353033,
-8.00795114489806));
#107542=CARTESIAN_POINT('Ctrl Pts',(-20.2366096474223,20.7022632248489,
-8.00844304711825));
#107543=CARTESIAN_POINT('Ctrl Pts',(-20.2340914542446,20.7047963003654,
-8.00865906350769));
#107544=CARTESIAN_POINT('Ctrl Pts',(-20.2286618069518,20.7102304609905,
-8.00912476054446));
#107545=CARTESIAN_POINT('Ctrl Pts',(-20.225748354315,20.7131294015686,-8.00937459675336));
#107546=CARTESIAN_POINT('Ctrl Pts',(-20.2176786507927,20.7211122788836,
-8.01006641244211));
#107547=CARTESIAN_POINT('Ctrl Pts',(-20.212504785718,20.7261782168353,-8.01050976324142));
#107548=CARTESIAN_POINT('Ctrl Pts',(-20.1839451609985,20.753856521646,-8.01295540519318));
#107549=CARTESIAN_POINT('Ctrl Pts',(-20.1600679338781,20.7759527773244,
-8.01499402291496));
#107550=CARTESIAN_POINT('Ctrl Pts',(-20.0137580453866,20.9052203256788,
-8.0273998941035));
#107551=CARTESIAN_POINT('Ctrl Pts',(-19.8798138343924,20.9985328676181,
-8.03835715738868));
#107552=CARTESIAN_POINT('Ctrl Pts',(-19.6336216446591,21.1308996988453,
-8.05661524271468));
#107553=CARTESIAN_POINT('Ctrl Pts',(-19.526323430212,21.1776126576731,-8.06405608414213));
#107554=CARTESIAN_POINT('Ctrl Pts',(-19.4021738965136,21.2198396724125,
-8.07206314263055));
#107555=CARTESIAN_POINT('Ctrl Pts',(-19.3885991768308,21.2243040304063,
-8.07293111877289));
#107556=CARTESIAN_POINT('Ctrl Pts',(-19.366922360117,21.2311905268723,-8.07430542749688));
#107557=CARTESIAN_POINT('Ctrl Pts',(-19.3588493389351,21.233702100081,-8.07481468814729));
#107558=CARTESIAN_POINT('Ctrl Pts',(-19.3445847674101,21.2380463564072,
-8.07571006634878));
#107559=CARTESIAN_POINT('Ctrl Pts',(-19.3383995131545,21.2398991890058,
-8.07609684002707));
#107560=CARTESIAN_POINT('Ctrl Pts',(-19.3255888911096,21.2436729119852,
-8.07689490880411));
#107561=CARTESIAN_POINT('Ctrl Pts',(-19.3189624102432,21.2455897777038,
-8.07730606852224));
#107562=CARTESIAN_POINT('Ctrl Pts',(-19.3019291031211,21.250426968723,-8.07835877822346));
#107563=CARTESIAN_POINT('Ctrl Pts',(-19.2915089853879,21.2533000672519,
-8.07899878690564));
#107564=CARTESIAN_POINT('Ctrl Pts',(-19.2479272749469,21.2649582753908,
-8.08165945088431));
#107565=CARTESIAN_POINT('Ctrl Pts',(-19.2145755250427,21.2730167803175,
-8.08365657747511));
#107566=CARTESIAN_POINT('Ctrl Pts',(-19.127178851698,21.2918978704387,-8.0888006502615));
#107567=CARTESIAN_POINT('Ctrl Pts',(-19.0728802726973,21.3014273158352,
-8.09190820756228));
#107568=CARTESIAN_POINT('Ctrl Pts',(-18.9099124879943,21.3235104553182,
-8.10105261517301));
#107569=CARTESIAN_POINT('Ctrl Pts',(-18.800578682725,21.3297764841732,-8.10694073608899));
#107570=CARTESIAN_POINT('Ctrl Pts',(-18.6455302129237,21.3266448901245,
-8.11538394594907));
#107571=CARTESIAN_POINT('Ctrl Pts',(-18.5998530274913,21.3242402979392,
-8.11788435240091));
#107572=CARTESIAN_POINT('Ctrl Pts',(-18.5315822066191,21.3184238939376,
-8.121683725345));
#107573=CARTESIAN_POINT('Ctrl Pts',(-18.5089067037586,21.3161226539018,
-8.12295602795445));
#107574=CARTESIAN_POINT('Ctrl Pts',(-18.4852456492105,21.3133347363886,
-8.12429840239874));
#107575=CARTESIAN_POINT('Ctrl Pts',(-18.4842180238449,21.3132128900864,
-8.12435673239391));
#107576=CARTESIAN_POINT('Ctrl Pts',(-18.4649310487697,21.3109116774326,
-8.12545205327248));
#107577=CARTESIAN_POINT('Ctrl Pts',(-18.4467012450516,21.3084953023214,
-8.12649667173703));
#107578=CARTESIAN_POINT('Ctrl Pts',(-18.3954025259099,21.3010143246308,
-8.12946827570211));
#107579=CARTESIAN_POINT('Ctrl Pts',(-18.3624204620127,21.2954031501119,
-8.13141652591858));
#107580=CARTESIAN_POINT('Ctrl Pts',(-18.3227886349005,21.287690199803,-8.13381814793919));
#107581=CARTESIAN_POINT('Ctrl Pts',(-18.3159965927483,21.2863337373251,
-8.13423189616548));
#107582=CARTESIAN_POINT('Ctrl Pts',(-18.304855544583,21.2840518098103,-8.13491430553586));
#107583=CARTESIAN_POINT('Ctrl Pts',(-18.3005025208339,21.2831459177625,
-8.13518187439928));
#107584=CARTESIAN_POINT('Ctrl Pts',(-18.2926676551979,21.2814896637643,
-8.13566520646445));
#107585=CARTESIAN_POINT('Ctrl Pts',(-18.2891848291454,21.2807442232738,
-8.13588068607341));
#107586=CARTESIAN_POINT('Ctrl Pts',(-18.2815902696258,21.2790986804165,
-8.13635192841704));
#107587=CARTESIAN_POINT('Ctrl Pts',(-18.2774793851383,21.2781951150224,
-8.13660788297164));
#107588=CARTESIAN_POINT('Ctrl Pts',(-18.2658602580979,21.2756049018854,
-8.13733374098581));
#107589=CARTESIAN_POINT('Ctrl Pts',(-18.2583585692817,21.2738895860056,
-8.13780524118772));
#107590=CARTESIAN_POINT('Ctrl Pts',(-18.2118556405573,21.2629892140187,
-8.14074514235477));
#107591=CARTESIAN_POINT('Ctrl Pts',(-18.1731150447937,21.2527399571674,
-8.14326888438847));
#107592=CARTESIAN_POINT('Ctrl Pts',(-17.9685915573466,21.1923712004236,
-8.15690935316512));
#107593=CARTESIAN_POINT('Ctrl Pts',(-17.8091349993931,21.1231483572091,
-8.16860034017371));
#107594=CARTESIAN_POINT('Ctrl Pts',(-17.5748943676725,20.9852296621986,
-8.18622209495736));
#107595=CARTESIAN_POINT('Ctrl Pts',(-17.4934949350718,20.929304034047,-8.19245943349971));
#107596=CARTESIAN_POINT('Ctrl Pts',(-17.4053697450291,20.8592187500021,
-8.19933147006765));
#107597=CARTESIAN_POINT('Ctrl Pts',(-17.3945430211814,20.8504323465081,
-8.20017811802275));
#107598=CARTESIAN_POINT('Ctrl Pts',(-17.3773696158958,20.8362116120886,
-8.20152511587853));
#107599=CARTESIAN_POINT('Ctrl Pts',(-17.3709670679166,20.8308456754649,
-8.20202821552975));
#107600=CARTESIAN_POINT('Ctrl Pts',(-17.3596847241826,20.8212757540045,
-8.20291645183421));
#107601=CARTESIAN_POINT('Ctrl Pts',(-17.3547920679314,20.8170871591606,
-8.20330221166024));
#107602=CARTESIAN_POINT('Ctrl Pts',(-17.344666695465,20.8083384559043,-8.20410177236088));
#107603=CARTESIAN_POINT('Ctrl Pts',(-17.3394371310998,20.8037748052531,
-8.20451542011653));
#107604=CARTESIAN_POINT('Ctrl Pts',(-17.3259758392404,20.7919105034922,
-8.20558203771492));
#107605=CARTESIAN_POINT('Ctrl Pts',(-17.3177783470846,20.7845711912914,
-8.20623338557506));
#107606=CARTESIAN_POINT('Ctrl Pts',(-17.2829809838188,20.7529245069529,
-8.20900657420588));
#107607=CARTESIAN_POINT('Ctrl Pts',(-17.2569458891753,20.7280032138624,
-8.21110227037802));
#107608=CARTESIAN_POINT('Ctrl Pts',(-17.1900041520504,20.6605671555438,
-8.21656087570482));
#107609=CARTESIAN_POINT('Ctrl Pts',(-17.1502155649188,20.6169856848495,
-8.21987777033214));
#107610=CARTESIAN_POINT('Ctrl Pts',(-17.0040346104367,20.4427773459455,
-8.23248460572176));
#107611=CARTESIAN_POINT('Ctrl Pts',(-16.9115655999521,20.3013123221957,
-8.24134744939338));
#107612=CARTESIAN_POINT('Ctrl Pts',(-16.8126538433843,20.1015551754427,
-8.25387130412168));
#107613=CARTESIAN_POINT('Ctrl Pts',(-16.7903660746532,20.0518006054982,
-8.25699617925251));
#107614=CARTESIAN_POINT('Ctrl Pts',(-16.7667528499304,19.9931153814201,
-8.26074974563898));
#107615=CARTESIAN_POINT('Ctrl Pts',(-16.7635317152814,19.9849641801932,
-8.26127259550564));
#107616=CARTESIAN_POINT('Ctrl Pts',(-16.758736153102,19.9726048321004,-8.26206796025164));
#107617=CARTESIAN_POINT('Ctrl Pts',(-16.7571243087456,19.9684111734145,
-8.26233828450779));
#107618=CARTESIAN_POINT('Ctrl Pts',(-16.7542575786825,19.9608810917377,
-8.2628245328397));
#107619=CARTESIAN_POINT('Ctrl Pts',(-16.7529977601694,19.9575466040421,
-8.26304015759751));
#107620=CARTESIAN_POINT('Ctrl Pts',(-16.7502814963103,19.9503019062624,
-8.26350930585135));
#107621=CARTESIAN_POINT('Ctrl Pts',(-16.7488282072439,19.9463906193554,
-8.26376300794614));
#107622=CARTESIAN_POINT('Ctrl Pts',(-16.7447856904949,19.9354115466325,
-8.26447627188808));
#107623=CARTESIAN_POINT('Ctrl Pts',(-16.7422226112388,19.9283342928819,
-8.26493734528075));
#107624=CARTESIAN_POINT('Ctrl Pts',(-16.7272663571117,19.8863384269095,
-8.26768033005309));
#107625=CARTESIAN_POINT('Ctrl Pts',(-16.7157547264623,19.8511152498446,
-8.27000951277372));
#107626=CARTESIAN_POINT('Ctrl Pts',(-16.6811834284812,19.7351081467683,
-8.2777327908292));
#107627=CARTESIAN_POINT('Ctrl Pts',(-16.6620070545219,19.6532540281286,
-8.28326092204806));
#107628=CARTESIAN_POINT('Ctrl Pts',(-16.6172146324318,19.3933020309549,
-8.30068485188907));
#107629=CARTESIAN_POINT('Ctrl Pts',(-16.6093739541459,19.212914346402,-8.31250730874657));
#107630=CARTESIAN_POINT('Ctrl Pts',(-16.6263355366115,19.0111193713292,
-8.32496771542771));
#107631=CARTESIAN_POINT('Ctrl Pts',(-16.628594135158,18.9885860554209,-8.32634975246745));
#107632=CARTESIAN_POINT('Ctrl Pts',(-16.6323116477244,18.9566673223458,
-8.32829481314576));
#107633=CARTESIAN_POINT('Ctrl Pts',(-16.6334727635477,18.9472494084905,
-8.32886716127869));
#107634=CARTESIAN_POINT('Ctrl Pts',(-16.6354657538434,18.931932808445,-8.32979552680643));
#107635=CARTESIAN_POINT('Ctrl Pts',(-16.6362592617004,18.926029342388,-8.33015275042749));
#107636=CARTESIAN_POINT('Ctrl Pts',(-16.637975400756,18.9136574886664,-8.33090016173763));
#107637=CARTESIAN_POINT('Ctrl Pts',(-16.6389030839445,18.9071898561725,
-8.33129018551736));
#107638=CARTESIAN_POINT('Ctrl Pts',(-16.6411871212474,18.8917741236501,
-8.3322181930552));
#107639=CARTESIAN_POINT('Ctrl Pts',(-16.6425709488715,18.8828301757122,
-8.33275530147617));
#107640=CARTESIAN_POINT('Ctrl Pts',(-16.6474566566296,18.8525396779709,
-8.33457010559597));
#107641=CARTESIAN_POINT('Ctrl Pts',(-16.6512284129043,18.8312375831703,
-8.33583924520943));
#107642=CARTESIAN_POINT('Ctrl Pts',(-16.6737782541512,18.7143464355662,
-8.34276958649708));
#107643=CARTESIAN_POINT('Ctrl Pts',(-16.6988112710497,18.6200782894915,
-8.34822624713029));
#107644=CARTESIAN_POINT('Ctrl Pts',(-16.7737993194569,18.4001273663881,
-8.36099710371439));
#107645=CARTESIAN_POINT('Ctrl Pts',(-16.8294586823472,18.2768584786398,
-8.36817945517728));
#107646=CARTESIAN_POINT('Ctrl Pts',(-16.9041964086709,18.1462230184113,
-8.37655369570066));
#107647=CARTESIAN_POINT('Ctrl Pts',(-16.9120732801524,18.1328004758076,
-8.37742396767121));
#107648=CARTESIAN_POINT('Ctrl Pts',(-16.9472976337008,18.0742649059864,
-8.38126790410149));
#107649=CARTESIAN_POINT('Ctrl Pts',(-16.9761757042415,18.0301000143669,
-8.38429629711212));
#107650=CARTESIAN_POINT('Ctrl Pts',(-17.0116955329246,17.9799712101822,
-8.38794237774091));
#107651=CARTESIAN_POINT('Ctrl Pts',(-17.0167645801836,17.9729099121094,
-8.38846097419108));
#107652=CARTESIAN_POINT('Ctrl Pts',(-17.0245101761043,17.9622591991466,
-8.38925112112448));
#107653=CARTESIAN_POINT('Ctrl Pts',(-17.0271549333267,17.9586466300419,
-8.38952052367901));
#107654=CARTESIAN_POINT('Ctrl Pts',(-17.0319252814881,17.9521738198729,
-8.39000579143878));
#107655=CARTESIAN_POINT('Ctrl Pts',(-17.034046650294,17.9493105343655,-8.39022136257886));
#107656=CARTESIAN_POINT('Ctrl Pts',(-17.0386747861549,17.9430966404029,
-8.39069118841527));
#107657=CARTESIAN_POINT('Ctrl Pts',(-17.0411842283435,17.9397481474907,
-8.39094562604249));
#107658=CARTESIAN_POINT('Ctrl Pts',(-17.0482684602618,17.930353420368,-8.391662994154));
#107659=CARTESIAN_POINT('Ctrl Pts',(-17.0528657740952,17.9243243623628,
-8.39212746371394));
#107660=CARTESIAN_POINT('Ctrl Pts',(-17.0807007083364,17.8882246263595,
-8.39493261631368));
#107661=CARTESIAN_POINT('Ctrl Pts',(-17.1047106885366,17.8587614259561,
-8.39732304757671));
#107662=CARTESIAN_POINT('Ctrl Pts',(-17.1867203120694,17.7634819342764,
-8.40535046610004));
#107663=CARTESIAN_POINT('Ctrl Pts',(-17.2480149309345,17.7006260651215,
-8.41113241175424));
#107664=CARTESIAN_POINT('Ctrl Pts',(-17.4423290221763,17.5246716669501,
-8.42845312280769));
#107665=CARTESIAN_POINT('Ctrl Pts',(-17.5856342033998,17.4239923843037,
-8.43990132062418));
#107666=CARTESIAN_POINT('Ctrl Pts',(-17.7600534528488,17.331199728219,-8.45206277306558));
#107667=CARTESIAN_POINT('Ctrl Pts',(-17.7805913041882,17.3207003244761,
-8.45347080372527));
#107668=CARTESIAN_POINT('Ctrl Pts',(-17.8098777285528,17.3063272237661,
-8.45544568632157));
#107669=CARTESIAN_POINT('Ctrl Pts',(-17.8184866945323,17.3021742485732,
-8.45602225603627));
#107670=CARTESIAN_POINT('Ctrl Pts',(-17.8325171624734,17.2955226907508,
-8.45695558888772));
#107671=CARTESIAN_POINT('Ctrl Pts',(-17.8379215538362,17.2929885172246,
-8.45731358410124));
#107672=CARTESIAN_POINT('Ctrl Pts',(-17.8492538994521,17.2877330184803,
-8.45806112192241));
#107673=CARTESIAN_POINT('Ctrl Pts',(-17.8551838658238,17.2850161609144,
-8.45845050714453));
#107674=CARTESIAN_POINT('Ctrl Pts',(-17.8693159695207,17.2786202922171,
-8.45937429077242));
#107675=CARTESIAN_POINT('Ctrl Pts',(-17.877529212119,17.2749660124574,-8.45990783498824));
#107676=CARTESIAN_POINT('Ctrl Pts',(-17.9052540260613,17.2628414989501,
-8.46169788147031));
#107677=CARTESIAN_POINT('Ctrl Pts',(-17.9248703083587,17.2546128641837,
-8.46294614647993));
#107678=CARTESIAN_POINT('Ctrl Pts',(-18.0885207382021,17.1888473888761,
-8.47321745326249));
#107679=CARTESIAN_POINT('Ctrl Pts',(-18.2383561212894,17.1470016270937,
-8.48166671119933));
#107680=CARTESIAN_POINT('Ctrl Pts',(-18.5257346406427,17.0998780267568,
-8.49748117395406));
#107681=CARTESIAN_POINT('Ctrl Pts',(-18.6618271134729,17.0908605546421,
-8.50483302257926));
#107682=CARTESIAN_POINT('Ctrl Pts',(-18.8134283353893,17.0954329492276,
-8.51372669283649));
#107683=CARTESIAN_POINT('Ctrl Pts',(-18.8290293538823,17.0960763142369,
-8.51465042055911));
#107684=CARTESIAN_POINT('Ctrl Pts',(-18.8503921865413,17.0971941306936,
-8.51592867720537));
#107685=CARTESIAN_POINT('Ctrl Pts',(-18.8561617258545,17.0975197173487,
-8.51627523879971));
#107686=CARTESIAN_POINT('Ctrl Pts',(-18.865332399465,17.0980749135176,-8.51682832773566));
#107687=CARTESIAN_POINT('Ctrl Pts',(-18.8687344859943,17.0982891257582,
-8.51703399783409));
#107688=CARTESIAN_POINT('Ctrl Pts',(-18.8757637449014,17.0987487703053,
-8.51745998154834));
#107689=CARTESIAN_POINT('Ctrl Pts',(-18.8793907968412,17.0989953285727,
-8.51768036000098));
#107690=CARTESIAN_POINT('Ctrl Pts',(-18.888038373376,17.0996055513629,-8.51820712741096));
#107691=CARTESIAN_POINT('Ctrl Pts',(-18.8930582554253,17.0999777811714,
-8.51851399292017));
#107692=CARTESIAN_POINT('Ctrl Pts',(-18.9100140911606,17.1012958970198,
-8.51955404132159));
#107693=CARTESIAN_POINT('Ctrl Pts',(-18.9219430788029,17.1023251207571,
-8.52029167527382));
#107694=CARTESIAN_POINT('Ctrl Pts',(-19.058975194832,17.1153201314184,-8.52882833096445));
#107695=CARTESIAN_POINT('Ctrl Pts',(-19.1827700137946,17.138300833222,-8.53713204906159));
#107696=CARTESIAN_POINT('Ctrl Pts',(-19.4646935637701,17.2170865602461,
-8.55647671210745));
#107697=CARTESIAN_POINT('Ctrl Pts',(-19.619747527816,17.2809545129042,-8.56741235140886));
#107698=CARTESIAN_POINT('Ctrl Pts',(-19.7862055411517,17.3738543308215,
-8.57915174424997));
#107699=CARTESIAN_POINT('Ctrl Pts',(-19.8065247159106,17.3856420860227,
-8.58058612436764));
#107700=CARTESIAN_POINT('Ctrl Pts',(-19.834737149007,17.4026427321543,-8.58258038378754));
#107701=CARTESIAN_POINT('Ctrl Pts',(-19.8427974910587,17.4075737032734,
-8.58315046283729));
#107702=CARTESIAN_POINT('Ctrl Pts',(-19.8563859001443,17.4160120486852,
-8.58411214211518));
#107703=CARTESIAN_POINT('Ctrl Pts',(-19.8619311463022,17.4194913662208,
-8.58450476711414));
#107704=CARTESIAN_POINT('Ctrl Pts',(-19.8728926162624,17.426440116179,-8.58528127060543));
#107705=CARTESIAN_POINT('Ctrl Pts',(-19.8783093421466,17.4299086207597,
-8.5856651778542));
#107706=CARTESIAN_POINT('Ctrl Pts',(-19.8891596012715,17.43692632237,-8.58643460602489));
#107707=CARTESIAN_POINT('Ctrl Pts',(-19.8945927894194,17.4404759259902,
-8.58682010627732));
#107708=CARTESIAN_POINT('Ctrl Pts',(-19.9138389949438,17.4531764930154,
-8.58818652430193));
#107709=CARTESIAN_POINT('Ctrl Pts',(-19.9275610394943,17.4624647261385,
-8.58916229315734));
#107710=CARTESIAN_POINT('Ctrl Pts',(-20.0449882486269,17.5439758706704,
-8.59752966848056));
#107711=CARTESIAN_POINT('Ctrl Pts',(-20.1421484798553,17.6251930698747,
-8.60454806203147));
#107712=CARTESIAN_POINT('Ctrl Pts',(-20.3274770907587,17.8106575464539,
-8.6188567048415));
#107713=CARTESIAN_POINT('Ctrl Pts',(-20.4139881948288,17.9157154158987,
-8.62609796880144));
#107714=CARTESIAN_POINT('Ctrl Pts',(-20.5158511784127,18.0669441804967,
-8.63641321351391));
#107715=CARTESIAN_POINT('Ctrl Pts',(-20.5405818680822,18.1064102163149,
-8.6390983240072));
#107716=CARTESIAN_POINT('Ctrl Pts',(-20.5678430828171,18.1532820306659,
-8.64231814207972));
#107717=CARTESIAN_POINT('Ctrl Pts',(-20.5716607533356,18.1599287813493,
-8.64277544070319));
#107718=CARTESIAN_POINT('Ctrl Pts',(-20.5777215519317,18.1706148857748,
-8.64351201608973));
#107719=CARTESIAN_POINT('Ctrl Pts',(-20.5799877389192,18.1746411751752,
-8.64378985066426));
#107720=CARTESIAN_POINT('Ctrl Pts',(-20.5839887627887,18.1818044752853,
-8.64428476126932));
#107721=CARTESIAN_POINT('Ctrl Pts',(-20.5857288325681,18.1849385101275,
-8.64450149778334));
#107722=CARTESIAN_POINT('Ctrl Pts',(-20.5894120814875,18.1916122852367,
-8.64496348701184));
#107723=CARTESIAN_POINT('Ctrl Pts',(-20.5913530655499,18.1951531146861,
-8.64520886806589));
#107724=CARTESIAN_POINT('Ctrl Pts',(-20.596590458459,18.2047725900186,-8.64587618405547));
#107725=CARTESIAN_POINT('Ctrl Pts',(-20.5998672000462,18.2108618069068,
-8.64629933750692));
#107726=CARTESIAN_POINT('Ctrl Pts',(-20.6163198486875,18.2417982766792,
-8.64845248001302));
#107727=CARTESIAN_POINT('Ctrl Pts',(-20.6290288278897,18.2668890126877,
-8.65020948010647));
#107728=CARTESIAN_POINT('Ctrl Pts',(-20.6647759863615,18.3410944524601,
-8.6554208437193));
#107729=CARTESIAN_POINT('Ctrl Pts',(-20.6864298666476,18.3908485600598,
-8.65893358048579));
#107730=CARTESIAN_POINT('Ctrl Pts',(-20.7117862945679,18.4558239130744,
-8.6634990956526));
#107731=CARTESIAN_POINT('Ctrl Pts',(-20.7172641108656,18.4703295411108,
-8.66451700717518));
#107732=CARTESIAN_POINT('Ctrl Pts',(-20.7225805936643,18.484889662309,-8.66553669489169));
#107733=CARTESIAN_POINT('',(-20.8507520319894,19.2105366956018,-7.68905625085211));
#107734=CARTESIAN_POINT('Ctrl Pts',(-20.7225806137986,18.4848897174502,
-8.44448866019381));
#107735=CARTESIAN_POINT('Ctrl Pts',(-20.6978226921706,18.417085798169,-8.44016253807091));
#107736=CARTESIAN_POINT('Ctrl Pts',(-20.6696011102778,18.350572196178,-8.435836415948));
#107737=CARTESIAN_POINT('Ctrl Pts',(-20.6380875635549,18.2857219064975,
-8.4315102938251));
#107738=CARTESIAN_POINT('Ctrl Pts',(-20.6065603427493,18.2208434775462,
-8.42718229454911));
#107739=CARTESIAN_POINT('Ctrl Pts',(-20.5717385521847,18.1576302317059,
-8.42285429527312));
#107740=CARTESIAN_POINT('Ctrl Pts',(-20.5338394211753,18.0964296531922,
-8.41852629599714));
#107741=CARTESIAN_POINT('Ctrl Pts',(-20.4958706676413,18.035116646275,-8.41419034597851));
#107742=CARTESIAN_POINT('Ctrl Pts',(-20.4548135633609,17.9758240998444,
-8.40985439595988));
#107743=CARTESIAN_POINT('Ctrl Pts',(-20.4109278137949,17.9188691601385,
-8.40551844594126));
#107744=CARTESIAN_POINT('Ctrl Pts',(-20.3707284188952,17.8666983726878,
-8.40154671095239));
#107745=CARTESIAN_POINT('Ctrl Pts',(-20.3281563085948,17.8164887934209,
-8.39757497596352));
#107746=CARTESIAN_POINT('Ctrl Pts',(-20.2834377820475,17.7684565657965,
-8.39360324097465));
#107747=CARTESIAN_POINT('Ctrl Pts',(-20.2340300954518,17.7153877052549,
-8.38921503204375));
#107748=CARTESIAN_POINT('Ctrl Pts',(-20.1817963672772,17.6647565409338,
-8.38482682311285));
#107749=CARTESIAN_POINT('Ctrl Pts',(-20.1270066890244,17.6168791249302,
-8.38043861418195));
#107750=CARTESIAN_POINT('Ctrl Pts',(-20.0722983277384,17.5690727669502,
-8.37605691808068));
#107751=CARTESIAN_POINT('Ctrl Pts',(-20.01504190713,17.5240123587826,-8.37167522197942));
#107752=CARTESIAN_POINT('Ctrl Pts',(-19.9555455237307,17.4819784462149,
-8.36729352587816));
#107753=CARTESIAN_POINT('Ctrl Pts',(-19.8961190533169,17.4399939268396,
-8.36291697861851));
#107754=CARTESIAN_POINT('Ctrl Pts',(-19.8344582408824,17.4010291152647,
-8.35854043135888));
#107755=CARTESIAN_POINT('Ctrl Pts',(-19.7709042257785,17.3653243441594,
-8.35416388409923));
#107756=CARTESIAN_POINT('Ctrl Pts',(-19.7073905157073,17.329642216501,-8.34979011238226));
#107757=CARTESIAN_POINT('Ctrl Pts',(-19.6419864047148,17.2972162628699,
-8.34541634066529));
#107758=CARTESIAN_POINT('Ctrl Pts',(-19.5750607832524,17.2682427431933,
-8.34104256894831));
#107759=CARTESIAN_POINT('Ctrl Pts',(-19.5081555274812,17.2392780402561,
-8.33667012818476));
#107760=CARTESIAN_POINT('Ctrl Pts',(-19.4397301228482,17.2137638770621,
-8.3322976874212));
#107761=CARTESIAN_POINT('Ctrl Pts',(-19.3701752330593,17.1918491703585,
-8.32792524665765));
#107762=CARTESIAN_POINT('Ctrl Pts',(-19.3006185647443,17.1699339032935,
-8.32355269409031));
#107763=CARTESIAN_POINT('Ctrl Pts',(-19.2299328146155,17.1516184185037,
-8.31918014152297));
#107764=CARTESIAN_POINT('Ctrl Pts',(-19.1585240564104,17.1370018501626,
-8.31480758895562));
#107765=CARTESIAN_POINT('Ctrl Pts',(-19.0870411875025,17.1223701121955,
-8.3104304983883));
#107766=CARTESIAN_POINT('Ctrl Pts',(-19.0148342859542,17.1114450521883,
-8.30605340782097));
#107767=CARTESIAN_POINT('Ctrl Pts',(-18.9423190546115,17.1042745381788,
-8.30167631725364));
#107768=CARTESIAN_POINT('Ctrl Pts',(-18.8697642200095,17.0971001080854,
-8.2972968361947));
#107769=CARTESIAN_POINT('Ctrl Pts',(-18.7969012025321,17.0936843291133,
-8.29291735513576));
#107770=CARTESIAN_POINT('Ctrl Pts',(-18.7241475303643,17.0940229267084,
-8.28853787407682));
#107771=CARTESIAN_POINT('Ctrl Pts',(-18.6512649028008,17.0943621244655,
-8.2841506304171));
#107772=CARTESIAN_POINT('Ctrl Pts',(-18.5784924896208,17.0984689605669,
-8.27976338675737));
#107773=CARTESIAN_POINT('Ctrl Pts',(-18.506243930902,17.1062871518924,-8.27537614309765));
#107774=CARTESIAN_POINT('Ctrl Pts',(-18.457121872828,17.1116027686346,-8.27239324016284));
#107775=CARTESIAN_POINT('Ctrl Pts',(-18.4082418439356,17.1186329436866,
-8.26941033722803));
#107776=CARTESIAN_POINT('Ctrl Pts',(-18.3597305432932,17.1273466282089,
-8.26642743429323));
#107777=CARTESIAN_POINT('Ctrl Pts',(-18.2883645862437,17.1401655060193,
-8.26203922536233));
#107778=CARTESIAN_POINT('Ctrl Pts',(-18.2175186632352,17.1566801162964,
-8.25765101643143));
#107779=CARTESIAN_POINT('Ctrl Pts',(-18.1476047194718,17.1768344278367,
-8.25326280750054));
#107780=CARTESIAN_POINT('Ctrl Pts',(-18.0777945395928,17.1969588270371,
-8.24888111139927));
#107781=CARTESIAN_POINT('Ctrl Pts',(-18.0089140527666,17.2207120714409,
-8.24449941529801));
#107782=CARTESIAN_POINT('Ctrl Pts',(-17.9413659204122,17.2479869547362,
-8.24011771919674));
#107783=CARTESIAN_POINT('Ctrl Pts',(-17.8738971624889,17.275229787873,-8.2357411719371));
#107784=CARTESIAN_POINT('Ctrl Pts',(-17.8077580939885,17.3059858596158,
-8.23136462467746));
#107785=CARTESIAN_POINT('Ctrl Pts',(-17.743335448913,17.3400984132725,-8.22698807741782));
#107786=CARTESIAN_POINT('Ctrl Pts',(-17.6789536597427,17.3741893332434,
-8.22261430570085));
#107787=CARTESIAN_POINT('Ctrl Pts',(-17.6162865594643,17.4116322864694,
-8.21824053398388));
#107788=CARTESIAN_POINT('Ctrl Pts',(-17.5556988450224,17.4522233262354,
-8.21386676226691));
#107789=CARTESIAN_POINT('Ctrl Pts',(-17.4951295676255,17.4928020140117,
-8.20949432150335));
#107790=CARTESIAN_POINT('Ctrl Pts',(-17.4366388203457,17.5365266181305,
-8.2051218807398));
#107791=CARTESIAN_POINT('Ctrl Pts',(-17.3805632774557,17.5831492580496,
-8.20074943997625));
#107792=CARTESIAN_POINT('Ctrl Pts',(-17.3244863007078,17.6297730901148,
-8.1963768874089));
#107793=CARTESIAN_POINT('Ctrl Pts',(-17.2708250206044,17.6792947951746,
-8.19200433484156));
#107794=CARTESIAN_POINT('Ctrl Pts',(-17.2198825933093,17.7314265889263,
-8.18763178227421));
#107795=CARTESIAN_POINT('Ctrl Pts',(-17.1688872960418,17.7836124870198,
-8.18325469170688));
#107796=CARTESIAN_POINT('Ctrl Pts',(-17.1206168232081,17.8384135364602,
-8.17887760113955));
#107797=CARTESIAN_POINT('Ctrl Pts',(-17.0753364363188,17.8955061070015,
-8.17450051057222));
#107798=CARTESIAN_POINT('Ctrl Pts',(-17.0300313201297,17.9526298579144,
-8.17012102951329));
#107799=CARTESIAN_POINT('Ctrl Pts',(-16.9877198211689,18.0120472284182,
-8.16574154845435));
#107800=CARTESIAN_POINT('Ctrl Pts',(-16.9486243453002,18.0734048296493,
-8.16136206739541));
#107801=CARTESIAN_POINT('Ctrl Pts',(-16.909459572963,18.1348711868168,-8.15697482373569));
#107802=CARTESIAN_POINT('Ctrl Pts',(-16.873522445187,18.1982842223064,-8.15258758007597));
#107803=CARTESIAN_POINT('Ctrl Pts',(-16.840989532304,18.2632656652873,-8.14820033641625));
#107804=CARTESIAN_POINT('Ctrl Pts',(-16.8188702864075,18.3074467849174,
-8.14521743348143));
#107805=CARTESIAN_POINT('Ctrl Pts',(-16.7983237185205,18.3523524542016,
-8.14223453054661));
#107806=CARTESIAN_POINT('Ctrl Pts',(-16.779392301285,18.3978593331261,-8.13925162761179));
#107807=CARTESIAN_POINT('Ctrl Pts',(-16.7515419099037,18.4648054245267,
-8.13486341868089));
#107808=CARTESIAN_POINT('Ctrl Pts',(-16.7270805292277,18.5333146794851,
-8.13047520975));
#107809=CARTESIAN_POINT('Ctrl Pts',(-16.7061840240079,18.6030103886487,
-8.1260870008191));
#107810=CARTESIAN_POINT('Ctrl Pts',(-16.6853185326665,18.6726026578242,
-8.12170530471783));
#107811=CARTESIAN_POINT('Ctrl Pts',(-16.6680075510804,18.7433774273515,
-8.11732360861657));
#107812=CARTESIAN_POINT('Ctrl Pts',(-16.654378888696,18.8149380939565,-8.1129419125153));
#107813=CARTESIAN_POINT('Ctrl Pts',(-16.6407662410746,18.8864146710833,
-8.10856536525566));
#107814=CARTESIAN_POINT('Ctrl Pts',(-16.6308274068038,18.9586748392569,
-8.10418881799602));
#107815=CARTESIAN_POINT('Ctrl Pts',(-16.6246399100932,19.0313085669594,
-8.09981227073638));
#107816=CARTESIAN_POINT('Ctrl Pts',(-16.618456337403,19.1038962314074,-8.09543849901941));
#107817=CARTESIAN_POINT('Ctrl Pts',(-16.6160194227851,19.1768565058774,
-8.09106472730244));
#107818=CARTESIAN_POINT('Ctrl Pts',(-16.6173550828665,19.2497723454648,
-8.08669095558546));
#107819=CARTESIAN_POINT('Ctrl Pts',(-16.618690336502,19.3226659965173,-8.08231851482191));
#107820=CARTESIAN_POINT('Ctrl Pts',(-16.6237958768595,19.3955147575249,
-8.07794607405836));
#107821=CARTESIAN_POINT('Ctrl Pts',(-16.6326455110292,19.4679013656683,
-8.07357363329481));
#107822=CARTESIAN_POINT('Ctrl Pts',(-16.641495371485,19.5402898247453,-8.06920108072745));
#107823=CARTESIAN_POINT('Ctrl Pts',(-16.6540894553073,19.6122156289261,
-8.0648285281601));
#107824=CARTESIAN_POINT('Ctrl Pts',(-16.670349874122,19.6832680996675,-8.06045597559275));
#107825=CARTESIAN_POINT('Ctrl Pts',(-16.6866271686126,19.754394311343,-8.05607888502542));
#107826=CARTESIAN_POINT('Ctrl Pts',(-16.7065782873149,19.8246449087061,
-8.0517017944581));
#107827=CARTESIAN_POINT('Ctrl Pts',(-16.7300746894323,19.8936216738912,
-8.04732470389077));
#107828=CARTESIAN_POINT('Ctrl Pts',(-16.7535839238069,19.9626361098477,
-8.04294522283183));
#107829=CARTESIAN_POINT('Ctrl Pts',(-16.7806421175113,20.0303748802481,
-8.03856574177288));
#107830=CARTESIAN_POINT('Ctrl Pts',(-16.8110725105125,20.096459694268,-8.03418626071394));
#107831=CARTESIAN_POINT('Ctrl Pts',(-16.841556841181,20.1626616431772,-8.02979901705422));
#107832=CARTESIAN_POINT('Ctrl Pts',(-16.8754250830337,20.2272033538502,
-8.0254117733945));
#107833=CARTESIAN_POINT('Ctrl Pts',(-16.9124547443363,20.2897316077547,
-8.02102452973478));
#107834=CARTESIAN_POINT('Ctrl Pts',(-16.9376313458523,20.3322447952014,
-8.01804162679997));
#107835=CARTESIAN_POINT('Ctrl Pts',(-16.9642684397432,20.3738277943096,
-8.01505872386516));
#107836=CARTESIAN_POINT('Ctrl Pts',(-16.992285306212,20.4143781306983,-8.01207582093036));
#107837=CARTESIAN_POINT('Ctrl Pts',(-17.033501486001,20.4740325519721,-8.00768761199946));
#107838=CARTESIAN_POINT('Ctrl Pts',(-17.0778664461833,20.5316834623514,
-8.00329940306856));
#107839=CARTESIAN_POINT('Ctrl Pts',(-17.1251586260628,20.5869790817843,
-7.99891119413766));
#107840=CARTESIAN_POINT('Ctrl Pts',(-17.1723806165062,20.6421926333496,
-7.99452949803641));
#107841=CARTESIAN_POINT('Ctrl Pts',(-17.2225208913246,20.6950574697366,
-7.99014780193515));
#107842=CARTESIAN_POINT('Ctrl Pts',(-17.2753151507576,20.7452514495971,
-7.9857661058339));
#107843=CARTESIAN_POINT('Ctrl Pts',(-17.3280473727344,20.7953864475367,
-7.98138955857426));
#107844=CARTESIAN_POINT('Ctrl Pts',(-17.3834270362631,20.8428564928137,
-7.97701301131462));
#107845=CARTESIAN_POINT('Ctrl Pts',(-17.4411513321099,20.8873744575526,
-7.97263646405498));
#107846=CARTESIAN_POINT('Ctrl Pts',(-17.4988390200472,20.9318641896452,
-7.96826269233801));
#107847=CARTESIAN_POINT('Ctrl Pts',(-17.5588680089998,20.9734052619584,
-7.96388892062104));
#107848=CARTESIAN_POINT('Ctrl Pts',(-17.6209016583803,21.0117501442131,
-7.95951514890407));
#107849=CARTESIAN_POINT('Ctrl Pts',(-17.6829164307129,21.0500833579914,
-7.95514270814051));
#107850=CARTESIAN_POINT('Ctrl Pts',(-17.7469342423152,21.0852220591674,
-7.95077026737696));
#107851=CARTESIAN_POINT('Ctrl Pts',(-17.8125900634642,21.1169624153831,
-7.9463978266134));
#107852=CARTESIAN_POINT('Ctrl Pts',(-17.8782475634396,21.1487035832032,
-7.94202527404607));
#107853=CARTESIAN_POINT('Ctrl Pts',(-17.9455427209574,21.1770460253878,
-7.93765272147873));
#107854=CARTESIAN_POINT('Ctrl Pts',(-18.0140880608545,21.2018329412273,
-7.9332801689114));
#107855=CARTESIAN_POINT('Ctrl Pts',(-18.082704539691,21.2266455818631,-7.92890307834407));
#107856=CARTESIAN_POINT('Ctrl Pts',(-18.152573336826,21.2478951643122,-7.92452598777674));
#107857=CARTESIAN_POINT('Ctrl Pts',(-18.2232900373585,21.2654742232646,
-7.92014889720942));
#107858=CARTESIAN_POINT('Ctrl Pts',(-18.2940453589056,21.2830628827936,
-7.91576941615048));
#107859=CARTESIAN_POINT('Ctrl Pts',(-18.3656490319724,21.2969769355905,
-7.91138993509155));
#107860=CARTESIAN_POINT('Ctrl Pts',(-18.4376872969879,21.307160247222,-7.90701045403262));
#107861=CARTESIAN_POINT('Ctrl Pts',(-18.5098532493447,21.317361608705,-7.9026232103729));
#107862=CARTESIAN_POINT('Ctrl Pts',(-18.5824548510264,21.3238189809293,
-7.89823596671317));
#107863=CARTESIAN_POINT('Ctrl Pts',(-18.6550746705894,21.3265282537412,
-7.89384872305345));
#107864=CARTESIAN_POINT('Ctrl Pts',(-18.7044491502636,21.3283702981885,
-7.89086582011861));
#107865=CARTESIAN_POINT('Ctrl Pts',(-18.7538320255725,21.328480806371,-7.88788291718377));
#107866=CARTESIAN_POINT('Ctrl Pts',(-18.8030934396838,21.3268721834252,
-7.88490001424892));
#107867=CARTESIAN_POINT('Ctrl Pts',(-18.8755629038515,21.3245057056244,
-7.88051180531802));
#107868=CARTESIAN_POINT('Ctrl Pts',(-18.9480521075247,21.3184071393707,
-7.87612359638712));
#107869=CARTESIAN_POINT('Ctrl Pts',(-19.020145332748,21.3085723702763,-7.87173538745622));
#107870=CARTESIAN_POINT('Ctrl Pts',(-19.092131559672,21.2987521976099,-7.86735369135494));
#107871=CARTESIAN_POINT('Ctrl Pts',(-19.1637225008059,21.2852068946333,
-7.86297199525365));
#107872=CARTESIAN_POINT('Ctrl Pts',(-19.2345042258083,21.267984326617,-7.85859029915237));
#107873=CARTESIAN_POINT('Ctrl Pts',(-19.3052027766504,21.2507819964888,
-7.85421375189273));
#107874=CARTESIAN_POINT('Ctrl Pts',(-19.3750935339405,21.2299110986508,
-7.84983720463309));
#107875=CARTESIAN_POINT('Ctrl Pts',(-19.4437711636792,21.2054708308746,
-7.84546065737346));
#107876=CARTESIAN_POINT('Ctrl Pts',(-19.5124052390632,21.181046062761,-7.84108688565648));
#107877=CARTESIAN_POINT('Ctrl Pts',(-19.5798272600416,21.1530565773996,
-7.83671311393951));
#107878=CARTESIAN_POINT('Ctrl Pts',(-19.645646875657,21.1216514528047,-7.83233934222254));
#107879=CARTESIAN_POINT('Ctrl Pts',(-19.7114464621423,21.0902558848947,
-7.82796690145899));
#107880=CARTESIAN_POINT('Ctrl Pts',(-19.7756441762378,21.0554469488639,
-7.82359446069543));
#107881=CARTESIAN_POINT('Ctrl Pts',(-19.8378710435217,21.0174212463527,
-7.81922201993188));
#107882=CARTESIAN_POINT('Ctrl Pts',(-19.9000995019534,20.97939457152,-7.81484946736454));
#107883=CARTESIAN_POINT('Ctrl Pts',(-19.9603566029528,20.9381512201346,
-7.81047691479719));
#107884=CARTESIAN_POINT('Ctrl Pts',(-20.0183007689806,20.8939321242391,
-7.80610436222985));
#107885=CARTESIAN_POINT('Ctrl Pts',(-20.0763050716495,20.8496671360979,
-7.80172727166252));
#107886=CARTESIAN_POINT('Ctrl Pts',(-20.1319912623925,20.8024205306336,
-7.79735018109519));
#107887=CARTESIAN_POINT('Ctrl Pts',(-20.185050077775,20.752474187844,-7.79297309052786));
#107888=CARTESIAN_POINT('Ctrl Pts',(-20.2381378705458,20.7025005675028,
-7.78859360946892));
#107889=CARTESIAN_POINT('Ctrl Pts',(-20.2885950971614,20.6498246228585,
-7.78421412840997));
#107890=CARTESIAN_POINT('Ctrl Pts',(-20.3361505972387,20.5947638757272,
-7.77983464735103));
#107891=CARTESIAN_POINT('Ctrl Pts',(-20.3837903891206,20.5396055337913,
-7.77544740369131));
#107892=CARTESIAN_POINT('Ctrl Pts',(-20.4285178872519,20.4820543293407,
-7.77106016003158));
#107893=CARTESIAN_POINT('Ctrl Pts',(-20.4701036879207,20.4224590314114,
-7.76667291637186));
#107894=CARTESIAN_POINT('Ctrl Pts',(-20.4983780251769,20.3819399714091,
-7.76369001343707));
#107895=CARTESIAN_POINT('Ctrl Pts',(-20.5252009588541,20.3404766042677,
-7.76070711050228));
#107896=CARTESIAN_POINT('Ctrl Pts',(-20.5505126306682,20.2981848336979,
-7.75772420756748));
#107897=CARTESIAN_POINT('Ctrl Pts',(-20.5890325091506,20.2338242543132,
-7.75318475796428));
#107898=CARTESIAN_POINT('Ctrl Pts',(-20.6241921153259,20.1673074236142,
-7.74864530836107));
#107899=CARTESIAN_POINT('Ctrl Pts',(-20.6557527999571,20.09900629269,-7.74410585875786));
#107900=CARTESIAN_POINT('Ctrl Pts',(-20.6876473131869,20.0299827163852,
-7.73951839377991));
#107901=CARTESIAN_POINT('Ctrl Pts',(-20.7158660149377,19.9591372097163,
-7.73493092880197));
#107902=CARTESIAN_POINT('Ctrl Pts',(-20.7402081049558,19.8868831552935,
-7.73034346382402));
#107903=CARTESIAN_POINT('Ctrl Pts',(-20.7642010194565,19.8156655503632,
-7.7258218038142));
#107904=CARTESIAN_POINT('Ctrl Pts',(-20.7844276391864,19.7430799630087,
-7.72130014380437));
#107905=CARTESIAN_POINT('Ctrl Pts',(-20.800742748614,19.6695448844458,-7.71677848379455));
#107906=CARTESIAN_POINT('Ctrl Pts',(-20.8174140154883,19.5944045413925,
-7.71215811633254));
#107907=CARTESIAN_POINT('Ctrl Pts',(-20.8300007712015,19.5182731789951,
-7.70753774887053));
#107908=CARTESIAN_POINT('Ctrl Pts',(-20.8384015048747,19.441615060829,-7.70291738140852));
#107909=CARTESIAN_POINT('Ctrl Pts',(-20.8468022385479,19.3649569426629,
-7.69829701394651));
#107910=CARTESIAN_POINT('Ctrl Pts',(-20.8510168371563,19.2877725479369,
-7.69367664648451));
#107911=CARTESIAN_POINT('Ctrl Pts',(-20.850999949394,19.2105371115439,-7.6890562790225));
#107912=CARTESIAN_POINT('Ctrl Pts',(-20.8476071281599,19.2105314192558,
-7.68905589350251));
#107913=CARTESIAN_POINT('Ctrl Pts',(-20.8480884203062,18.9629933058656,
-7.67422393940026));
#107914=CARTESIAN_POINT('Ctrl Pts',(-20.8073981352126,18.7156059215239,
-7.65939198529801));
#107915=CARTESIAN_POINT('Ctrl Pts',(-20.7249099383763,18.4840591618169,
-7.64456003119576));
#107916=CARTESIAN_POINT('Origin',(-18.734,19.211,0.));
#107917=CARTESIAN_POINT('',(-20.7225806151895,18.4848897212595,-6.84500607926505));
#107918=CARTESIAN_POINT('',(-20.7225806056755,18.4848896952038,-7.06814847058112));
#107919=CARTESIAN_POINT('',(-20.7225806137986,18.4848897174502,0.));
#107920=CARTESIAN_POINT('',(-20.8510002458083,19.2120354932906,-7.10922378494469));
#107921=CARTESIAN_POINT('Ctrl Pts',(-20.7225806056755,18.4848896952038,
-7.06814847058112));
#107922=CARTESIAN_POINT('Ctrl Pts',(-20.7469467821702,18.5516207492762,
-7.07223678875001));
#107923=CARTESIAN_POINT('Ctrl Pts',(-20.7679438661329,18.6195503552378,
-7.07621988970315));
#107924=CARTESIAN_POINT('Ctrl Pts',(-20.829084658028,18.8595719529904,-7.0898896347857));
#107925=CARTESIAN_POINT('Ctrl Pts',(-20.8510858772448,19.0354726805544,
-7.09915343889004));
#107926=CARTESIAN_POINT('Ctrl Pts',(-20.8509997481128,19.212032710241,-7.10922276175899));
#107927=CARTESIAN_POINT('Ctrl Pts',(-20.8509997467294,19.212035542177,-7.10922292326604));
#107928=CARTESIAN_POINT('Ctrl Pts',(-20.8509866388109,19.238832577368,-7.11075117535696));
#107929=CARTESIAN_POINT('Ctrl Pts',(-20.8504647358669,19.2656259780468,
-7.11229812416721));
#107930=CARTESIAN_POINT('Ctrl Pts',(-20.8488772351525,19.306881542247,-7.1147189423379));
#107931=CARTESIAN_POINT('Ctrl Pts',(-20.8481713907108,19.3213553130007,
-7.1155756299352));
#107932=CARTESIAN_POINT('Ctrl Pts',(-20.847039981172,19.34051107497,-7.11672056384823));
#107933=CARTESIAN_POINT('Ctrl Pts',(-20.8467473097919,19.3452009113002,
-7.11700175783987));
#107934=CARTESIAN_POINT('Ctrl Pts',(-20.8462061821906,19.3534311774479,
-7.11749684192021));
#107935=CARTESIAN_POINT('Ctrl Pts',(-20.8459644307084,19.3569720500464,
-7.11771036402102));
#107936=CARTESIAN_POINT('Ctrl Pts',(-20.8454718256778,19.3639296117368,
-7.11813097919925));
#107937=CARTESIAN_POINT('Ctrl Pts',(-20.8452215797129,19.3673463399483,
-7.11833803869449));
#107938=CARTESIAN_POINT('Ctrl Pts',(-20.8446669325148,19.374674968951,-7.11878326863147));
#107939=CARTESIAN_POINT('Ctrl Pts',(-20.8443599503591,19.3785866188367,
-7.11902158000591));
#107940=CARTESIAN_POINT('Ctrl Pts',(-20.8435234723322,19.3888783451667,
-7.11965031160079));
#107941=CARTESIAN_POINT('Ctrl Pts',(-20.8429759114186,19.3952568550261,
-7.12004172511595));
#107942=CARTESIAN_POINT('Ctrl Pts',(-20.8405832027644,19.4217202366947,
-7.12167260083017));
#107943=CARTESIAN_POINT('Ctrl Pts',(-20.8384800652699,19.4417799699492,
-7.12292549519722));
#107944=CARTESIAN_POINT('Ctrl Pts',(-20.835585736007,19.4660383587798,-7.12445837341481));
#107945=CARTESIAN_POINT('Ctrl Pts',(-20.8350679509523,19.4702694257601,
-7.12472638862714));
#107946=CARTESIAN_POINT('Ctrl Pts',(-20.8313092230471,19.500232926735,-7.1266289285973));
#107947=CARTESIAN_POINT('Ctrl Pts',(-20.8276085458607,19.5259044409515,
-7.12828252494956));
#107948=CARTESIAN_POINT('Ctrl Pts',(-20.7949769851179,19.7261438788488,
-7.1413336803723));
#107949=CARTESIAN_POINT('Ctrl Pts',(-20.7447340062298,19.8965335727698,
-7.15327774337597));
#107950=CARTESIAN_POINT('Ctrl Pts',(-20.6502651860484,20.1127161683493,
-7.16848804445987));
#107951=CARTESIAN_POINT('Ctrl Pts',(-20.6244119201432,20.1657293204335,
-7.17223080315733));
#107952=CARTESIAN_POINT('Ctrl Pts',(-20.5792508989512,20.2492848789387,
-7.17814298236814));
#107953=CARTESIAN_POINT('Ctrl Pts',(-20.5613178022045,20.2805308643735,
-7.18035723787088));
#107954=CARTESIAN_POINT('Ctrl Pts',(-20.5368774061374,20.3207040517759,
-7.18321038315292));
#107955=CARTESIAN_POINT('Ctrl Pts',(-20.5310863590702,20.330057929371,-7.18387517373648));
#107956=CARTESIAN_POINT('Ctrl Pts',(-20.5215233221819,20.345238749928,-7.18495497962293));
#107957=CARTESIAN_POINT('Ctrl Pts',(-20.5177951807465,20.3510929453834,
-7.18537160435052));
#107958=CARTESIAN_POINT('Ctrl Pts',(-20.5105519342274,20.3623443046225,
-7.18617279265389));
#107959=CARTESIAN_POINT('Ctrl Pts',(-20.5070408606974,20.3677439606527,
-7.18655750017841));
#107960=CARTESIAN_POINT('Ctrl Pts',(-20.498919027194,20.3801106120571,-7.18743910752061));
#107961=CARTESIAN_POINT('Ctrl Pts',(-20.4942915398638,20.3870665344756,
-7.18793537409213));
#107962=CARTESIAN_POINT('Ctrl Pts',(-20.4818301475165,20.4055598561801,
-7.18925592976821));
#107963=CARTESIAN_POINT('Ctrl Pts',(-20.4739231320461,20.4170476702888,
-7.19007745492741));
#107964=CARTESIAN_POINT('Ctrl Pts',(-20.4095513678279,20.5086202508339,
-7.19663791284082));
#107965=CARTESIAN_POINT('Ctrl Pts',(-20.3476984772763,20.5847799811123,
-7.20215962191543));
#107966=CARTESIAN_POINT('Ctrl Pts',(-20.1873374477826,20.7563905983615,
-7.21511375898675));
#107967=CARTESIAN_POINT('Ctrl Pts',(-20.0844177080016,20.8470902846918,
-7.22239522681411));
#107968=CARTESIAN_POINT('Ctrl Pts',(-19.9318268842307,20.9572926963362,
-7.23282452956406));
#107969=CARTESIAN_POINT('Ctrl Pts',(-19.889107549375,20.9858389406645,-7.23571235750914));
#107970=CARTESIAN_POINT('Ctrl Pts',(-19.8300638695438,21.0222585378053,
-7.23972036859023));
#107971=CARTESIAN_POINT('Ctrl Pts',(-19.8146125671854,21.031519138202,-7.24077074177687));
#107972=CARTESIAN_POINT('Ctrl Pts',(-19.791573920485,21.0449305179197,-7.24234197176213));
#107973=CARTESIAN_POINT('Ctrl Pts',(-19.7840758999984,21.0492340277016,
-7.24285411880012));
#107974=CARTESIAN_POINT('Ctrl Pts',(-19.770452897438,21.0569424418053,-7.24378643146881));
#107975=CARTESIAN_POINT('Ctrl Pts',(-19.7643369253056,21.0603631131528,
-7.24420564019099));
#107976=CARTESIAN_POINT('Ctrl Pts',(-19.7546742301547,21.0657046622724,
-7.24486915771922));
#107977=CARTESIAN_POINT('Ctrl Pts',(-19.751138744273,21.0676459120229,-7.24511218495754));
#107978=CARTESIAN_POINT('Ctrl Pts',(-19.747588675693,21.0695819854432,-7.24535648936914));
#107979=CARTESIAN_POINT('Ctrl Pts',(-19.7475795859075,21.0695869425827,
-7.24535711490102));
#107980=CARTESIAN_POINT('Ctrl Pts',(-19.7475613507176,21.0695968870199,
-7.24535836979594));
#107981=CARTESIAN_POINT('Ctrl Pts',(-19.7475522053045,21.0696018743214,
-7.2453589991596));
#107982=CARTESIAN_POINT('Ctrl Pts',(-19.7475338597622,21.0696118785872,
-7.24536026165599));
#107983=CARTESIAN_POINT('Ctrl Pts',(-19.7475246581378,21.0696168963658,
-7.24536089489164));
#107984=CARTESIAN_POINT('Ctrl Pts',(-19.7475061984414,21.0696269625269,
-7.24536216525126));
#107985=CARTESIAN_POINT('Ctrl Pts',(-19.7474969416186,21.0696320102271,
-7.24536280228928));
#107986=CARTESIAN_POINT('Ctrl Pts',(-19.74747837093,21.0696421365528,-7.24536408029467));
#107987=CARTESIAN_POINT('Ctrl Pts',(-19.7474690572325,21.0696472150854,
-7.24536472125048));
#107988=CARTESIAN_POINT('Ctrl Pts',(-19.7474503730712,21.0696574029218,
-7.24536600707248));
#107989=CARTESIAN_POINT('Ctrl Pts',(-19.7474410022956,21.0696625123943,
-7.24536665196016));
#107990=CARTESIAN_POINT('Ctrl Pts',(-19.7474222031634,21.0696727625515,
-7.24536794570202));
#107991=CARTESIAN_POINT('Ctrl Pts',(-19.7474127753466,21.0696779029406,
-7.24536859451908));
#107992=CARTESIAN_POINT('Ctrl Pts',(-19.7473938621929,21.0696882148942,
-7.24536989611561));
#107993=CARTESIAN_POINT('Ctrl Pts',(-19.7473843762638,21.0696933867804,
-7.24537054893585));
#107994=CARTESIAN_POINT('Ctrl Pts',(-19.7473653458116,21.0697037623103,
-7.2453718586127));
#107995=CARTESIAN_POINT('Ctrl Pts',(-19.7473558022532,21.0697089654268,
-7.24537251540296));
#107996=CARTESIAN_POINT('Ctrl Pts',(-19.7473366566343,21.0697194033637,
-7.24537383301358));
#107997=CARTESIAN_POINT('Ctrl Pts',(-19.7473270539974,21.0697246384972,
-7.24537449387365));
#107998=CARTESIAN_POINT('Ctrl Pts',(-19.7473077898938,21.0697351406431,
-7.24537581964653));
#107999=CARTESIAN_POINT('Ctrl Pts',(-19.747298128484,21.0697404076234,-7.24537648455546));
#108000=CARTESIAN_POINT('Ctrl Pts',(-19.7472787461405,21.0697509738377,
-7.24537781847392));
#108001=CARTESIAN_POINT('Ctrl Pts',(-19.7472690253539,21.0697562729904,
-7.24537848747334));
#108002=CARTESIAN_POINT('Ctrl Pts',(-19.7472495617317,21.0697668831173,
-7.24537982699377));
#108003=CARTESIAN_POINT('Ctrl Pts',(-19.747239762086,21.0697722250598,-7.24538050142478));
#108004=CARTESIAN_POINT('Ctrl Pts',(-19.747220120423,21.0697829318393,-7.24538185320671));
#108005=CARTESIAN_POINT('Ctrl Pts',(-19.7472102800833,21.0697882957617,
-7.24538253044237));
#108006=CARTESIAN_POINT('Ctrl Pts',(-19.7471905368017,21.0697990575273,
-7.24538388922641));
#108007=CARTESIAN_POINT('Ctrl Pts',(-19.7471806358372,21.0698044542912,
-7.24538457063869));
#108008=CARTESIAN_POINT('Ctrl Pts',(-19.7471607708919,21.0698152819621,
-7.24538593780454));
#108009=CARTESIAN_POINT('Ctrl Pts',(-19.7471508087519,21.0698207118643,
-7.24538662343144));
#108010=CARTESIAN_POINT('Ctrl Pts',(-19.7471307895991,21.0698316231706,
-7.24538800121905));
#108011=CARTESIAN_POINT('Ctrl Pts',(-19.7471207816009,21.0698370778576,
-7.24538869000625));
#108012=CARTESIAN_POINT('Ctrl Pts',(-19.7441075652915,21.07147934817,-7.24559607133871));
#108013=CARTESIAN_POINT('Ctrl Pts',(-19.7411004588033,21.0731088485091,
-7.24580323311674));
#108014=CARTESIAN_POINT('Ctrl Pts',(-19.734048189569,21.0769082749406,-7.2462895287151));
#108015=CARTESIAN_POINT('Ctrl Pts',(-19.7299999213996,21.0790723293297,
-7.24656903072244));
#108016=CARTESIAN_POINT('Ctrl Pts',(-19.7175117266943,21.0856959230251,
-7.24743224548494));
#108017=CARTESIAN_POINT('Ctrl Pts',(-19.7090487868861,21.0901114857038,
-7.24801862673343));
#108018=CARTESIAN_POINT('Ctrl Pts',(-19.5959279689524,21.148162679678,-7.25587224861653));
#108019=CARTESIAN_POINT('Ctrl Pts',(-19.4870191423013,21.193038039962,-7.26360090159983));
#108020=CARTESIAN_POINT('Ctrl Pts',(-19.2704614072204,21.2618342266719,
-7.27860966937119));
#108021=CARTESIAN_POINT('Ctrl Pts',(-19.1635296367042,21.2868659915252,
-7.28586175390677));
#108022=CARTESIAN_POINT('Ctrl Pts',(-18.9798958472266,21.3150480880672,
-7.29780669591059));
#108023=CARTESIAN_POINT('Ctrl Pts',(-18.9040832937476,21.3225295485691,
-7.302598333006));
#108024=CARTESIAN_POINT('Ctrl Pts',(-18.8090892881317,21.3267527863396,
-7.30842436700041));
#108025=CARTESIAN_POINT('Ctrl Pts',(-18.790143078176,21.3273402953087,-7.30957773020232));
#108026=CARTESIAN_POINT('Ctrl Pts',(-18.7626111758836,21.3278240449663,
-7.31124168769252));
#108027=CARTESIAN_POINT('Ctrl Pts',(-18.7540303813472,21.3279226305993,
-7.31175858917514));
#108028=CARTESIAN_POINT('Ctrl Pts',(-18.738995838723,21.3280039413551,-7.31266134982074));
#108029=CARTESIAN_POINT('Ctrl Pts',(-18.732542372347,21.3280093346203,-7.31304791387815));
#108030=CARTESIAN_POINT('Ctrl Pts',(-18.7200192406795,21.327962536269,-7.31379626560532));
#108031=CARTESIAN_POINT('Ctrl Pts',(-18.7139496327782,21.3279137501448,
-7.31415815610573));
#108032=CARTESIAN_POINT('Ctrl Pts',(-18.699453270723,21.3277348791519,-7.31502057352149));
#108033=CARTESIAN_POINT('Ctrl Pts',(-18.6910268771331,21.3275805770049,
-7.31552033889434));
#108034=CARTESIAN_POINT('Ctrl Pts',(-18.6606992749911,21.3268440386015,
-7.31731370092195));
#108035=CARTESIAN_POINT('Ctrl Pts',(-18.6388060191357,21.3259721394975,
-7.31859824488434));
#108036=CARTESIAN_POINT('Ctrl Pts',(-18.4297009203736,21.3143908780171,
-7.3307809302873));
#108037=CARTESIAN_POINT('Ctrl Pts',(-18.2446857031687,21.2791944941734,
-7.34080119373469));
#108038=CARTESIAN_POINT('Ctrl Pts',(-17.9918550085426,21.1952207225491,
-7.35533055634334));
#108039=CARTESIAN_POINT('Ctrl Pts',(-17.9184496379319,21.1661948069355,
-7.35967215678778));
#108040=CARTESIAN_POINT('Ctrl Pts',(-17.8144380101076,21.118188605362,-7.36622721649198));
#108041=CARTESIAN_POINT('Ctrl Pts',(-17.7824203921183,21.102417071965,-7.36830359405264));
#108042=CARTESIAN_POINT('Ctrl Pts',(-17.7442251037883,21.0823872097441,
-7.37087033802637));
#108043=CARTESIAN_POINT('Ctrl Pts',(-17.7376497520927,21.0788947009194,
-7.37131548093427));
#108044=CARTESIAN_POINT('Ctrl Pts',(-17.7274341054552,21.0733993562359,
-7.3720123985891));
#108045=CARTESIAN_POINT('Ctrl Pts',(-17.7237809778512,21.0714203258339,
-7.37226268586176));
#108046=CARTESIAN_POINT('Ctrl Pts',(-17.7170029557306,21.0677225778187,
-7.37272910290817));
#108047=CARTESIAN_POINT('Ctrl Pts',(-17.7138765700374,21.0660067132131,
-7.37294505074972));
#108048=CARTESIAN_POINT('Ctrl Pts',(-17.7068004432007,21.0620998005357,
-7.37343565337955));
#108049=CARTESIAN_POINT('Ctrl Pts',(-17.7028533888527,21.0599040176485,
-7.37371060783005));
#108050=CARTESIAN_POINT('Ctrl Pts',(-17.6926708524161,21.0541966306698,
-7.37442322724189));
#108051=CARTESIAN_POINT('Ctrl Pts',(-17.6864461541182,21.050666042944,-7.37486206785098));
#108052=CARTESIAN_POINT('Ctrl Pts',(-17.6481280501512,21.0286748589315,
-7.37758278292947));
#108053=CARTESIAN_POINT('Ctrl Pts',(-17.6165076871889,21.009407721105,-7.37991175355753));
#108054=CARTESIAN_POINT('Ctrl Pts',(-17.442243393115,20.8968533354313,-7.39315500204117));
#108055=CARTESIAN_POINT('Ctrl Pts',(-17.3107668824149,20.7874349907261,
-7.40465479597926));
#108056=CARTESIAN_POINT('Ctrl Pts',(-17.1285733358706,20.5942356621574,
-7.42191011089756));
#108057=CARTESIAN_POINT('Ctrl Pts',(-17.0680484040015,20.5207118646229,
-7.42795239755897));
#108058=CARTESIAN_POINT('Ctrl Pts',(-17.0002336088481,20.4259894318504,
-7.43510796054048));
#108059=CARTESIAN_POINT('Ctrl Pts',(-16.9880630700075,20.4084345525163,
-7.43640986189084));
#108060=CARTESIAN_POINT('Ctrl Pts',(-16.9711422664415,20.3832212629625,
-7.43824622619549));
#108061=CARTESIAN_POINT('Ctrl Pts',(-16.9661722933924,20.3757125318183,
-7.43878896937054));
#108062=CARTESIAN_POINT('Ctrl Pts',(-16.9576834984331,20.3627079779575,
-7.43972192179025));
#108063=CARTESIAN_POINT('Ctrl Pts',(-16.9541419315327,20.357227219107,-7.44011298005118));
#108064=CARTESIAN_POINT('Ctrl Pts',(-16.9474110858534,20.3467044699221,
-7.44085975392969));
#108065=CARTESIAN_POINT('Ctrl Pts',(-16.9442176736913,20.3416652098244,
-7.44121562091924));
#108066=CARTESIAN_POINT('Ctrl Pts',(-16.9359727271505,20.3285320813027,
-7.44213855489813));
#108067=CARTESIAN_POINT('Ctrl Pts',(-16.9309544943303,20.3204173856874,
-7.44270438797607));
#108068=CARTESIAN_POINT('Ctrl Pts',(-16.9140481035296,20.2926613110696,
-7.44462502750829));
#108069=CARTESIAN_POINT('Ctrl Pts',(-16.9024244075849,20.2728601637084,
-7.44597017547181));
#108070=CARTESIAN_POINT('Ctrl Pts',(-16.8045469022421,20.099733511415,-7.45752710287622));
#108071=CARTESIAN_POINT('Ctrl Pts',(-16.7373941875307,19.9364022466313,
-7.46698362266903));
#108072=CARTESIAN_POINT('Ctrl Pts',(-16.6684626516087,19.6829753194227,
-7.48127480216599));
#108073=CARTESIAN_POINT('Ctrl Pts',(-16.6508703309531,19.5980060005061,
-7.48602197005629));
#108074=CARTESIAN_POINT('Ctrl Pts',(-16.6331668456332,19.4748441830829,
-7.49312667492237));
#108075=CARTESIAN_POINT('Ctrl Pts',(-16.6287970218653,19.4373486677181,
-7.49531931382054));
#108076=CARTESIAN_POINT('Ctrl Pts',(-16.6247572804446,19.3922219998179,
-7.49801499248867));
#108077=CARTESIAN_POINT('Ctrl Pts',(-16.6241229869961,19.3846814592724,
-7.49846733096744));
#108078=CARTESIAN_POINT('Ctrl Pts',(-16.6232010055168,19.3729694050171,
-7.49917307734983));
#108079=CARTESIAN_POINT('Ctrl Pts',(-16.6228852191966,19.3688000787462,
-7.49942493610065));
#108080=CARTESIAN_POINT('Ctrl Pts',(-16.6223231612413,19.3610754137424,
-7.49989276282739));
#108081=CARTESIAN_POINT('Ctrl Pts',(-16.6220735147062,19.357520378419,-7.5001085392746));
#108082=CARTESIAN_POINT('Ctrl Pts',(-16.6215302107451,19.34949358185,-7.50059679894941));
#108083=CARTESIAN_POINT('Ctrl Pts',(-16.6212417766759,19.3450215342786,
-7.50086956966399));
#108084=CARTESIAN_POINT('Ctrl Pts',(-16.6204344445541,19.3318533619991,
-7.50167487299511));
#108085=CARTESIAN_POINT('Ctrl Pts',(-16.6199550301464,19.3231550342996,
-7.50220953737669));
#108086=CARTESIAN_POINT('Ctrl Pts',(-16.6169292109334,19.2613111660761,
-7.50602903476624));
#108087=CARTESIAN_POINT('Ctrl Pts',(-16.6163337223535,19.2080936523045,
-7.50941043539998));
#108088=CARTESIAN_POINT('Ctrl Pts',(-16.6182284982312,19.136597479866,-7.51403235991408));
#108089=CARTESIAN_POINT('Ctrl Pts',(-16.6189517616592,19.1182869752344,
-7.51522308339859));
#108090=CARTESIAN_POINT('Ctrl Pts',(-16.6224277275562,19.0520911377894,
-7.5195484362301));
#108091=CARTESIAN_POINT('Ctrl Pts',(-16.6265698190564,19.0042941889997,
-7.5227104157986));
#108092=CARTESIAN_POINT('Ctrl Pts',(-16.6454711166344,18.8480959323211,
-7.53310371964198));
#108093=CARTESIAN_POINT('Ctrl Pts',(-16.6670072456871,18.7406844904373,
-7.54033607612409));
#108094=CARTESIAN_POINT('Ctrl Pts',(-16.7117292009486,18.5823942610658,
-7.55090879469441));
#108095=CARTESIAN_POINT('Ctrl Pts',(-16.7287734952871,18.5299773533292,
-7.55439753703905));
#108096=CARTESIAN_POINT('Ctrl Pts',(-16.7597165677077,18.4461010208939,
-7.55995455183979));
#108097=CARTESIAN_POINT('Ctrl Pts',(-16.7723691943367,18.4142125014765,
-7.56206125347214));
#108098=CARTESIAN_POINT('Ctrl Pts',(-16.7900208471462,18.3726976268708,
-7.56479760346392));
#108099=CARTESIAN_POINT('Ctrl Pts',(-16.7943261005433,18.3627836443009,
-7.56545058933261));
#108100=CARTESIAN_POINT('Ctrl Pts',(-16.8015031399717,18.3465970455908,
-7.56651606645575));
#108101=CARTESIAN_POINT('Ctrl Pts',(-16.8043299557075,18.3403048159528,
-7.56693008702831));
#108102=CARTESIAN_POINT('Ctrl Pts',(-16.8098622357212,18.3281497556809,
-7.56772959970173));
#108103=CARTESIAN_POINT('Ctrl Pts',(-16.8125638640162,18.3222852726665,
-7.5681152181177));
#108104=CARTESIAN_POINT('Ctrl Pts',(-16.8188649922172,18.3087703254852,
-7.56900364962267));
#108105=CARTESIAN_POINT('Ctrl Pts',(-16.8224835929839,18.3011288484176,
-7.56950579659309));
#108106=CARTESIAN_POINT('Ctrl Pts',(-16.8323412323096,18.2806306405874,
-7.57085244874572));
#108107=CARTESIAN_POINT('Ctrl Pts',(-16.8386648996876,18.2678149247873,
-7.57169401222917));
#108108=CARTESIAN_POINT('Ctrl Pts',(-16.8978944681167,18.1507802428592,
-7.57937831199596));
#108109=CARTESIAN_POINT('Ctrl Pts',(-16.9592192411624,18.0510396631901,
-7.58590412118604));
#108110=CARTESIAN_POINT('Ctrl Pts',(-17.1249845837826,17.8256123045543,
-7.60122216395494));
#108111=CARTESIAN_POINT('Ctrl Pts',(-17.236311721042,17.7059592805319,-7.60983082559518));
#108112=CARTESIAN_POINT('Ctrl Pts',(-17.3848200802793,17.579299529788,-7.62104054326569));
#108113=CARTESIAN_POINT('Ctrl Pts',(-17.4098779647989,17.5589002877034,
-7.62292525659317));
#108114=CARTESIAN_POINT('Ctrl Pts',(-17.4410979515934,17.534651137863,-7.62527904786693));
#108115=CARTESIAN_POINT('Ctrl Pts',(-17.4468272626404,17.5302479197882,
-7.62571122740489));
#108116=CARTESIAN_POINT('Ctrl Pts',(-17.4558478258553,17.5233884082339,
-7.62639222513861));
#108117=CARTESIAN_POINT('Ctrl Pts',(-17.4591239364024,17.5209121659685,
-7.62663966420562));
#108118=CARTESIAN_POINT('Ctrl Pts',(-17.4652633386587,17.5162997179251,
-7.62710361602306));
#108119=CARTESIAN_POINT('Ctrl Pts',(-17.4681248394151,17.5141612218448,
-7.62731996452228));
#108120=CARTESIAN_POINT('Ctrl Pts',(-17.4746722116452,17.5092939286056,
-7.62781522246919));
#108121=CARTESIAN_POINT('Ctrl Pts',(-17.4783615335456,17.506569868669,-7.62809445534763));
#108122=CARTESIAN_POINT('Ctrl Pts',(-17.4897393120993,17.4982259236788,
-7.62895603151567));
#108123=CARTESIAN_POINT('Ctrl Pts',(-17.4974567391075,17.4926460050014,
-7.62954102893509));
#108124=CARTESIAN_POINT('Ctrl Pts',(-17.6026931037089,17.417633166598,-7.637523314598));
#108125=CARTESIAN_POINT('Ctrl Pts',(-17.7058820850413,17.356549460309,-7.64539832406016));
#108126=CARTESIAN_POINT('Ctrl Pts',(-17.9117679230947,17.2571600545062,
-7.66050172347273));
#108127=CARTESIAN_POINT('Ctrl Pts',(-18.0133882175354,17.2174408067252,
-7.66770223878746));
#108128=CARTESIAN_POINT('Ctrl Pts',(-18.189357192284,17.1638859145967,-7.6795201694923));
#108129=CARTESIAN_POINT('Ctrl Pts',(-18.2622094568914,17.145878286301,-7.68423782880869));
#108130=CARTESIAN_POINT('Ctrl Pts',(-18.354336922749,17.1282377886458,-7.68998408675162));
#108131=CARTESIAN_POINT('Ctrl Pts',(-18.3728492830438,17.1249480647135,
-7.69112801922012));
#108132=CARTESIAN_POINT('Ctrl Pts',(-18.3998438808234,17.1205211447916,
-7.69278094959314));
#108133=CARTESIAN_POINT('Ctrl Pts',(-18.4082926746177,17.119188130447,-7.6932961380045));
#108134=CARTESIAN_POINT('Ctrl Pts',(-18.4231256089149,17.1169398998958,
-7.69419692106731));
#108135=CARTESIAN_POINT('Ctrl Pts',(-18.4295062413988,17.1160025913426,
-7.69458321121145));
#108136=CARTESIAN_POINT('Ctrl Pts',(-18.4419084710015,17.1142385734645,
-7.69533176838538));
#108137=CARTESIAN_POINT('Ctrl Pts',(-18.4479295348826,17.1134086119331,
-7.69569413478422));
#108138=CARTESIAN_POINT('Ctrl Pts',(-18.4623385252913,17.1114856292067,
-7.69655885604421));
#108139=CARTESIAN_POINT('Ctrl Pts',(-18.4707296339782,17.1104169220098,
-7.69706043993987));
#108140=CARTESIAN_POINT('Ctrl Pts',(-18.5010717403946,17.1067371647947,
-7.6988671635793));
#108141=CARTESIAN_POINT('Ctrl Pts',(-18.5230573802345,17.1044196148271,
-7.70016307062361));
#108142=CARTESIAN_POINT('Ctrl Pts',(-18.7299483776857,17.085882405688,-7.71224409602855));
#108143=CARTESIAN_POINT('Ctrl Pts',(-18.9161909189968,17.0937013233405,
-7.72217233217738));
#108144=CARTESIAN_POINT('Ctrl Pts',(-19.2068116659795,17.1445758292433,
-7.73825630792358));
#108145=CARTESIAN_POINT('Ctrl Pts',(-19.3129451810829,17.1717658806178,
-7.74428770586997));
#108146=CARTESIAN_POINT('Ctrl Pts',(-19.4276538344826,17.2108318754326,
-7.7514399859801));
#108147=CARTESIAN_POINT('Ctrl Pts',(-19.438788686742,17.214728209541,-7.75214113270838));
#108148=CARTESIAN_POINT('Ctrl Pts',(-19.4545988887945,17.2204093145448,
-7.75314726774578));
#108149=CARTESIAN_POINT('Ctrl Pts',(-19.4593016035648,17.2221179979071,
-7.75344788229311));
#108150=CARTESIAN_POINT('Ctrl Pts',(-19.4674057351831,17.2250951165373,
-7.75396831740386));
#108151=CARTESIAN_POINT('Ctrl Pts',(-19.4708100630542,17.2263556718151,
-7.7541876688923));
#108152=CARTESIAN_POINT('Ctrl Pts',(-19.4774126379573,17.2288198046164,
-7.75461453976269));
#108153=CARTESIAN_POINT('Ctrl Pts',(-19.4806112190219,17.2300223715317,
-7.75482199283272));
#108154=CARTESIAN_POINT('Ctrl Pts',(-19.4892507942977,17.2332944796223,
-7.75538408958011));
#108155=CARTESIAN_POINT('Ctrl Pts',(-19.4946861394802,17.235378709625,-7.75573959985214));
#108156=CARTESIAN_POINT('Ctrl Pts',(-19.514929688888,17.2432371974404,-7.75707052048708));
#108157=CARTESIAN_POINT('Ctrl Pts',(-19.5296808860076,17.2491555823059,
-7.75805405065918));
#108158=CARTESIAN_POINT('Ctrl Pts',(-19.6585622906279,17.3025572023171,
-7.76675921292675));
#108159=CARTESIAN_POINT('Ctrl Pts',(-19.7683864980642,17.3597819736637,
-7.77493889589455));
#108160=CARTESIAN_POINT('Ctrl Pts',(-20.0135027475799,17.5161539252156,
-7.7941521040843));
#108161=CARTESIAN_POINT('Ctrl Pts',(-20.1433088144144,17.6224472075079,
-7.80506970155752));
#108162=CARTESIAN_POINT('Ctrl Pts',(-20.2740376721806,17.7582693134469,
-7.81664817056723));
#108163=CARTESIAN_POINT('Ctrl Pts',(-20.2885731903803,17.7738344816468,
-7.81794610161462));
#108164=CARTESIAN_POINT('Ctrl Pts',(-20.3089101469849,17.7962816847784,
-7.81977788786208));
#108165=CARTESIAN_POINT('Ctrl Pts',(-20.3149060267143,17.8029850778136,
-7.82031996724489));
#108166=CARTESIAN_POINT('Ctrl Pts',(-20.3251770012896,17.8146163474709,
-7.82125213696267));
#108167=CARTESIAN_POINT('Ctrl Pts',(-20.329472334899,17.8195261107251,-7.82164307255232));
#108168=CARTESIAN_POINT('Ctrl Pts',(-20.3376537913389,17.8289655808528,
-7.82238985596887));
#108169=CARTESIAN_POINT('Ctrl Pts',(-20.3415435812567,17.8334920132112,
-7.82274585399512));
#108170=CARTESIAN_POINT('Ctrl Pts',(-20.3516099216603,17.845306620592,-7.82366965506387));
#108171=CARTESIAN_POINT('Ctrl Pts',(-20.3577564167394,17.8526203149127,
-7.82423621950626));
#108172=CARTESIAN_POINT('Ctrl Pts',(-20.3785534625371,17.8777095209664,
-7.82616204714698));
#108173=CARTESIAN_POINT('Ctrl Pts',(-20.3929636359234,17.8956828106609,
-7.82751157974486));
#108174=CARTESIAN_POINT('Ctrl Pts',(-20.514233917635,18.0521031367659,-7.83901212718583));
#108175=CARTESIAN_POINT('Ctrl Pts',(-20.6038503418906,18.2030609311729,
-7.84841818174308));
#108176=CARTESIAN_POINT('Ctrl Pts',(-20.6913710393355,18.4033523037698,
-7.86031012484889));
#108177=CARTESIAN_POINT('Ctrl Pts',(-20.7076100910747,18.4438903116821,
-7.86269368616636));
#108178=CARTESIAN_POINT('Ctrl Pts',(-20.72258060468,18.4848896924774,-7.86510589144174));
#108179=CARTESIAN_POINT('',(-20.8523540255571,19.2092594247491,-6.88905704671363));
#108180=CARTESIAN_POINT('Ctrl Pts',(-20.7249099383763,18.4840591618169,
-7.64456003119576));
#108181=CARTESIAN_POINT('Ctrl Pts',(-20.6989346215926,18.4111456946262,
-7.6398894877592));
#108182=CARTESIAN_POINT('Ctrl Pts',(-20.3954319387082,17.6922647742514,
-7.59282700876215));
#108183=CARTESIAN_POINT('Ctrl Pts',(-19.0148744805716,16.7235434527702,
-7.5033725942046));
#108184=CARTESIAN_POINT('Ctrl Pts',(-16.7944747214404,17.6284159605188,
-7.37619678752319));
#108185=CARTESIAN_POINT('Ctrl Pts',(-16.3534690248723,19.9852110982479,
-7.24902098084175));
#108186=CARTESIAN_POINT('Ctrl Pts',(-18.0964527455682,21.6317156062949,
-7.12184517416031));
#108187=CARTESIAN_POINT('Ctrl Pts',(-20.2927766547169,21.0898254884639,
-7.00185719611761));
#108188=CARTESIAN_POINT('Ctrl Pts',(-20.8471440721213,19.7934638825817,
-6.92426115363537));
#108189=CARTESIAN_POINT('Ctrl Pts',(-20.8523540255571,19.2092594247491,
-6.88905704671363));
#108190=CARTESIAN_POINT('Ctrl Pts',(-20.8509992391718,19.2092051891481,
-6.88983567993721));
#108191=CARTESIAN_POINT('Ctrl Pts',(-20.8509308802699,19.1285751086996,
-6.88542685664988));
#108192=CARTESIAN_POINT('Ctrl Pts',(-20.8462561258519,19.0480199742941,
-6.88096330535665));
#108193=CARTESIAN_POINT('Ctrl Pts',(-20.834275194884,18.9443612817674,-6.87493026745674));
#108194=CARTESIAN_POINT('Ctrl Pts',(-20.8311546079904,18.920837034468,-6.87354153241672));
#108195=CARTESIAN_POINT('Ctrl Pts',(-20.8267567249006,18.8914788094755,
-6.87177828995945));
#108196=CARTESIAN_POINT('Ctrl Pts',(-20.8258491620947,18.8855901323302,
-6.87142309733171));
#108197=CARTESIAN_POINT('Ctrl Pts',(-20.824284219736,18.8757132293002,-6.87082467057525));
#108198=CARTESIAN_POINT('Ctrl Pts',(-20.8236402485044,18.8717228727096,
-6.87058216746203));
#108199=CARTESIAN_POINT('Ctrl Pts',(-20.8224405319189,18.8644218499878,
-6.87013708432283));
#108200=CARTESIAN_POINT('Ctrl Pts',(-20.8218883302108,18.8611106037104,
-6.86993470344753));
#108201=CARTESIAN_POINT('Ctrl Pts',(-20.8207318334646,18.8542759683693,
-6.86951587247673));
#108202=CARTESIAN_POINT('Ctrl Pts',(-20.8201264940997,18.8507528216931,
-6.86929936162679));
#108203=CARTESIAN_POINT('Ctrl Pts',(-20.8187199415165,18.8426889554922,
-6.8688024187287));
#108204=CARTESIAN_POINT('Ctrl Pts',(-20.8179128176727,18.8381493228197,
-6.86852165476489));
#108205=CARTESIAN_POINT('Ctrl Pts',(-20.8153705414134,18.824116554734,-6.86765073281342));
#108206=CARTESIAN_POINT('Ctrl Pts',(-20.8135853303695,18.8146327756965,
-6.86705783825151));
#108207=CARTESIAN_POINT('Ctrl Pts',(-20.7945684265934,18.7172735616643,
-6.86092934697766));
#108208=CARTESIAN_POINT('Ctrl Pts',(-20.7718441214467,18.6305728922017,
-6.85512350878007));
#108209=CARTESIAN_POINT('Ctrl Pts',(-20.7369695777151,18.525244321258,-6.84783211541534));
#108210=CARTESIAN_POINT('Ctrl Pts',(-20.7299277512409,18.5050111446256,
-6.84642004455659));
#108211=CARTESIAN_POINT('Ctrl Pts',(-20.7225806151895,18.4848897212595,
-6.84500607926505));
#108212=CARTESIAN_POINT('Origin',(-18.734,19.211,0.));
#108213=CARTESIAN_POINT('',(-20.7225806138063,18.4848897174713,-6.04247212253779));
#108214=CARTESIAN_POINT('',(-20.7225804911066,18.4848893814367,-6.26710637686285));
#108215=CARTESIAN_POINT('',(-20.7225806137986,18.4848897174502,0.));
#108216=CARTESIAN_POINT('Ctrl Pts',(-20.7225804911066,18.4848893814367,
-6.26710637686285));
#108217=CARTESIAN_POINT('Ctrl Pts',(-20.7522829247855,18.5662346732453,
-6.27277686239517));
#108218=CARTESIAN_POINT('Ctrl Pts',(-20.7769957136057,18.6494073289697,
-6.27836339991924));
#108219=CARTESIAN_POINT('Ctrl Pts',(-20.8065479247142,18.7771762058336,
-6.2865811338612));
#108220=CARTESIAN_POINT('Ctrl Pts',(-20.8151860535273,18.8207141299219,
-6.2893203645065));
#108221=CARTESIAN_POINT('Ctrl Pts',(-20.8243855577728,18.8761611051668,
-6.29273465623541));
#108222=CARTESIAN_POINT('Ctrl Pts',(-20.8262235206868,18.8878442882777,
-6.29344996453055));
#108223=CARTESIAN_POINT('Ctrl Pts',(-20.8290114867732,18.9065880921723,
-6.29459112400719));
#108224=CARTESIAN_POINT('Ctrl Pts',(-20.8300239035339,18.913639045797,-6.29501894449509));
#108225=CARTESIAN_POINT('Ctrl Pts',(-20.8318772340533,18.9270264694107,
-6.2958285191774));
#108226=CARTESIAN_POINT('Ctrl Pts',(-20.8327250735366,18.9333618860314,
-6.29621048826961));
#108227=CARTESIAN_POINT('Ctrl Pts',(-20.8345859303218,18.9477627962086,
-6.29707616430485));
#108228=CARTESIAN_POINT('Ctrl Pts',(-20.835581216702,18.9558305101549,-6.29755930657332));
#108229=CARTESIAN_POINT('Ctrl Pts',(-20.8380346045802,18.9767062766664,
-6.29880485697251));
#108230=CARTESIAN_POINT('Ctrl Pts',(-20.8394222487224,18.989522390211,-6.2995650439401));
#108231=CARTESIAN_POINT('Ctrl Pts',(-20.8476032826374,19.0721247104989,
-6.3044370202131));
#108232=CARTESIAN_POINT('Ctrl Pts',(-20.85104361841,19.1422033440889,-6.30844168028271));
#108233=CARTESIAN_POINT('Ctrl Pts',(-20.8508787727464,19.4047165711849,
-6.3231406661448));
#108234=CARTESIAN_POINT('Ctrl Pts',(-20.8245352152959,19.5961656074274,
-6.3331749947728));
#108235=CARTESIAN_POINT('Ctrl Pts',(-20.759294768958,19.8293426961447,-6.34683371733216));
#108236=CARTESIAN_POINT('Ctrl Pts',(-20.744197911464,19.8767853283336,-6.34969721589345));
#108237=CARTESIAN_POINT('Ctrl Pts',(-20.7248154872869,19.9310025717403,
-6.35311512618809));
#108238=CARTESIAN_POINT('Ctrl Pts',(-20.7221455108881,19.9383427190911,
-6.35358099542427));
#108239=CARTESIAN_POINT('Ctrl Pts',(-20.7178168244118,19.9500409666448,
-6.35432874286635));
#108240=CARTESIAN_POINT('Ctrl Pts',(-20.7161841991077,19.9544087321618,
-6.35460910856059));
#108241=CARTESIAN_POINT('Ctrl Pts',(-20.7132689666539,19.9621299811691,
-6.35510688388085));
#108242=CARTESIAN_POINT('Ctrl Pts',(-20.7119922426185,19.9654856386655,
-6.35532393996009));
#108243=CARTESIAN_POINT('Ctrl Pts',(-20.7092701406778,19.972585833281,-6.35578476004516));
#108244=CARTESIAN_POINT('Ctrl Pts',(-20.7078226709785,19.9763294539083,
-6.35602864303979));
#108245=CARTESIAN_POINT('Ctrl Pts',(-20.7038921036952,19.9864098403162,
-6.35668776167519));
#108246=CARTESIAN_POINT('Ctrl Pts',(-20.7013891043818,19.9927387221509,
-6.35710416642735));
#108247=CARTESIAN_POINT('Ctrl Pts',(-20.6888792570119,20.0239294822189,
-6.35916872648583));
#108248=CARTESIAN_POINT('Ctrl Pts',(-20.6784319275977,20.0486106350645,
-6.36084135417825));
#108249=CARTESIAN_POINT('Ctrl Pts',(-20.6469617713902,20.1191931528088,
-6.36572421461722));
#108250=CARTESIAN_POINT('Ctrl Pts',(-20.6247626534134,20.1645478225075,
-6.36898505356392));
#108251=CARTESIAN_POINT('Ctrl Pts',(-20.5384183076348,20.3260626716198,
-6.38094758587727));
#108252=CARTESIAN_POINT('Ctrl Pts',(-20.4650106877013,20.4369262161604,
-6.38981579055469));
#108253=CARTESIAN_POINT('Ctrl Pts',(-20.3168836997383,20.6205484449742,
-6.40514171561398));
#108254=CARTESIAN_POINT('Ctrl Pts',(-20.2462642120733,20.6960623089784,
-6.41168265810236));
#108255=CARTESIAN_POINT('Ctrl Pts',(-20.1600892182026,20.7756583478519,
-6.41884330918656));
#108256=CARTESIAN_POINT('Ctrl Pts',(-20.1496786641039,20.7850839045917,
-6.41969611750575));
#108257=CARTESIAN_POINT('Ctrl Pts',(-20.1329049473183,20.7999695468413,
-6.4210510100854));
#108258=CARTESIAN_POINT('Ctrl Pts',(-20.1266019393969,20.8054965079818,
-6.42155589508113));
#108259=CARTESIAN_POINT('Ctrl Pts',(-20.1153950600402,20.8152064170283,
-6.42244619581993));
#108260=CARTESIAN_POINT('Ctrl Pts',(-20.1105046337667,20.8194046552351,
-6.42283224426577));
#108261=CARTESIAN_POINT('Ctrl Pts',(-20.1003178001555,20.8280691594151,
-6.42363134648645));
#108262=CARTESIAN_POINT('Ctrl Pts',(-20.0950184819654,20.8325318963423,
-6.4240442523738));
#108263=CARTESIAN_POINT('Ctrl Pts',(-20.081291059947,20.8439775228058,-6.4251067288252));
#108264=CARTESIAN_POINT('Ctrl Pts',(-20.0728304727572,20.8509212670814,
-6.42575470158249));
#108265=CARTESIAN_POINT('Ctrl Pts',(-20.0366931626524,20.8801136864495,
-6.42849390558301));
#108266=CARTESIAN_POINT('Ctrl Pts',(-20.0085118697073,20.9017305183268,
-6.4305597982846));
#108267=CARTESIAN_POINT('Ctrl Pts',(-19.9330683160028,20.9566416482939,
-6.43592260490661));
#108268=CARTESIAN_POINT('Ctrl Pts',(-19.8849623786337,20.9887277411595,
-6.43917558827396));
#108269=CARTESIAN_POINT('Ctrl Pts',(-19.6972065164932,21.103138197676,-6.45137510084861));
#108270=CARTESIAN_POINT('Ctrl Pts',(-19.5495978239829,21.1712929665874,
-6.45992613101447));
#108271=CARTESIAN_POINT('Ctrl Pts',(-19.3750774393533,21.2287161915827,
-6.47018702923805));
#108272=CARTESIAN_POINT('Ctrl Pts',(-19.3543836773646,21.2351746354237,
-6.4714067492847));
#108273=CARTESIAN_POINT('Ctrl Pts',(-19.2933193433325,21.2532082341672,
-6.47502442112291));
#108274=CARTESIAN_POINT('Ctrl Pts',(-19.2527016856321,21.2639005409562,
-6.47745420047644));
#108275=CARTESIAN_POINT('Ctrl Pts',(-19.2045508740802,21.2750557614865,
-6.48039068188202));
#108276=CARTESIAN_POINT('Ctrl Pts',(-19.1972969151105,21.2766960755133,
-6.48083455017466));
#108277=CARTESIAN_POINT('Ctrl Pts',(-19.1855407958701,21.2792894107184,
-6.48155652699095));
#108278=CARTESIAN_POINT('Ctrl Pts',(-19.1810438352741,21.2802660498957,
-6.48183331769278));
#108279=CARTESIAN_POINT('Ctrl Pts',(-19.1730488257041,21.2819751088501,
-6.48232657289057));
#108280=CARTESIAN_POINT('Ctrl Pts',(-19.1695520699089,21.2827133409351,
-6.48254270135557));
#108281=CARTESIAN_POINT('Ctrl Pts',(-19.1620432162948,21.2842787525061,
-6.48300767415887));
#108282=CARTESIAN_POINT('Ctrl Pts',(-19.1580306418605,21.2851031302024,
-6.48325666897805));
#108283=CARTESIAN_POINT('Ctrl Pts',(-19.1469792033555,21.2873402224293,
-6.48394384159974));
#108284=CARTESIAN_POINT('Ctrl Pts',(-19.1399355826728,21.2887287698348,
-6.4843833611645));
#108285=CARTESIAN_POINT('Ctrl Pts',(-19.1018130747293,21.2960428182941,
-6.48677006437656));
#108286=CARTESIAN_POINT('Ctrl Pts',(-19.0706131410091,21.3013065221611,
-6.4887515819924));
#108287=CARTESIAN_POINT('Ctrl Pts',(-18.8775474781523,21.3294441723526,
-6.50113876062034));
#108288=CARTESIAN_POINT('Ctrl Pts',(-18.7136045527413,21.3342040473118,
-6.51214901648214));
#108289=CARTESIAN_POINT('Ctrl Pts',(-18.4341372787239,21.309921658899,-6.53047401822961));
#108290=CARTESIAN_POINT('Ctrl Pts',(-18.3185530455791,21.2901347868,-6.53793076980914));
#108291=CARTESIAN_POINT('Ctrl Pts',(-18.1913415451304,21.2573174426433,
-6.54595263466364));
#108292=CARTESIAN_POINT('Ctrl Pts',(-18.1775384217965,21.2536071091668,
-6.54682080307756));
#108293=CARTESIAN_POINT('Ctrl Pts',(-18.1556307484283,21.2474796839016,
-6.54819535772543));
#108294=CARTESIAN_POINT('Ctrl Pts',(-18.1475014632004,21.2451533776193,
-6.54870467365861));
#108295=CARTESIAN_POINT('Ctrl Pts',(-18.1331892997412,21.2409648257023,
-6.54960011616502));
#108296=CARTESIAN_POINT('Ctrl Pts',(-18.1270006362122,21.2391228919689,
-6.549986899162));
#108297=CARTESIAN_POINT('Ctrl Pts',(-18.1142184291863,21.2352547721593,
-6.55078495567323));
#108298=CARTESIAN_POINT('Ctrl Pts',(-18.1076261601405,21.2332246147748,
-6.55119609396212));
#108299=CARTESIAN_POINT('Ctrl Pts',(-18.0907312374964,21.2279311068824,
-6.55224868361479));
#108300=CARTESIAN_POINT('Ctrl Pts',(-18.080443356312,21.2246209948174,-6.55288859436772));
#108301=CARTESIAN_POINT('Ctrl Pts',(-18.0376199801715,21.210479859638,-6.55554830669822));
#108302=CARTESIAN_POINT('Ctrl Pts',(-18.0053236369473,21.1989375733158,
-6.55754460104756));
#108303=CARTESIAN_POINT('Ctrl Pts',(-17.9219258491713,21.1668265721188,
-6.56268604595992));
#108304=CARTESIAN_POINT('Ctrl Pts',(-17.8713205893471,21.1450390082726,
-6.56579186038222));
#108305=CARTESIAN_POINT('Ctrl Pts',(-17.7229738117296,21.0741870079356,
-6.57493322723091));
#108306=CARTESIAN_POINT('Ctrl Pts',(-17.6281227950019,21.0195011125469,
-6.580820040185));
#108307=CARTESIAN_POINT('Ctrl Pts',(-17.5024504865063,20.9334467406348,
-6.58911240233665));
#108308=CARTESIAN_POINT('Ctrl Pts',(-17.4677299316055,20.9080848247028,
-6.59146229245138));
#108309=CARTESIAN_POINT('Ctrl Pts',(-17.3741856982365,20.8352849509247,
-6.59802420181248));
#108310=CARTESIAN_POINT('Ctrl Pts',(-17.3170978473414,20.7857324389769,
-6.60229302295449));
#108311=CARTESIAN_POINT('Ctrl Pts',(-17.2559602780968,20.7266443209607,
-6.6073321514166));
#108312=CARTESIAN_POINT('Ctrl Pts',(-17.2491784944956,20.7200010657329,
-6.60789803232228));
#108313=CARTESIAN_POINT('Ctrl Pts',(-17.2391914686884,20.7100855322071,
-6.60874209085317));
#108314=CARTESIAN_POINT('Ctrl Pts',(-17.2359516876903,20.7068479973701,
-6.60901759838665));
#108315=CARTESIAN_POINT('Ctrl Pts',(-17.2302041607973,20.7010670561246,
-6.60950944674124));
#108316=CARTESIAN_POINT('Ctrl Pts',(-17.227692320267,20.6985277918404,-6.60972545880299));
#108317=CARTESIAN_POINT('Ctrl Pts',(-17.2223034932822,20.6930524850478,
-6.61019118541858));
#108318=CARTESIAN_POINT('Ctrl Pts',(-17.2194286705741,20.6901144594914,
-6.61044105573938));
#108319=CARTESIAN_POINT('Ctrl Pts',(-17.2115115303713,20.681975978684,-6.61113305984481));
#108320=CARTESIAN_POINT('Ctrl Pts',(-17.2064873748197,20.6767580449853,
-6.6115765661542));
#108321=CARTESIAN_POINT('Ctrl Pts',(-17.1790222527096,20.6479390440077,
-6.61402463751384));
#108322=CARTESIAN_POINT('Ctrl Pts',(-17.1571027199689,20.6238497121559,
-6.61606561252066));
#108323=CARTESIAN_POINT('Ctrl Pts',(-17.0290696329091,20.4764507184679,
-6.62847227844776));
#108324=CARTESIAN_POINT('Ctrl Pts',(-16.9369045195771,20.3417523362035,
-6.63942738463181));
#108325=CARTESIAN_POINT('Ctrl Pts',(-16.8066265838216,20.0944949328792,
-6.65768271341527));
#108326=CARTESIAN_POINT('Ctrl Pts',(-16.7608185099317,19.9868184022987,
-6.66512287719615));
#108327=CARTESIAN_POINT('Ctrl Pts',(-16.7196357893792,19.862329416315,-6.67312930487364));
#108328=CARTESIAN_POINT('Ctrl Pts',(-16.7152852966763,19.8487179187452,
-6.67399727271548));
#108329=CARTESIAN_POINT('Ctrl Pts',(-16.7085806013527,19.8269843648363,
-6.67537157082266));
#108330=CARTESIAN_POINT('Ctrl Pts',(-16.7061367258244,19.8188906337728,
-6.67588082908637));
#108331=CARTESIAN_POINT('Ctrl Pts',(-16.7019120767193,19.8045902300333,
-6.67677620451176));
#108332=CARTESIAN_POINT('Ctrl Pts',(-16.700111102041,19.7983896843884,-6.67716297778781));
#108333=CARTESIAN_POINT('Ctrl Pts',(-16.6964447762704,19.7855479037243,
-6.67796104709484));
#108334=CARTESIAN_POINT('Ctrl Pts',(-16.6945834592252,19.7789055893083,
-6.67837220773847));
#108335=CARTESIAN_POINT('Ctrl Pts',(-16.6898890402123,19.7618322907801,
-6.67942492262433));
#108336=CARTESIAN_POINT('Ctrl Pts',(-16.6871032755738,19.7513884108513,
-6.68006493553586));
#108337=CARTESIAN_POINT('Ctrl Pts',(-16.6758102297431,19.7077099292253,
-6.68272564062173));
#108338=CARTESIAN_POINT('Ctrl Pts',(-16.6680311486553,19.6742912540351,
-6.68472280316241));
#108339=CARTESIAN_POINT('Ctrl Pts',(-16.6498821999752,19.5867375488995,
-6.68986698947393));
#108340=CARTESIAN_POINT('Ctrl Pts',(-16.6408076278669,19.5323596874423,
-6.69297462206998));
#108341=CARTESIAN_POINT('Ctrl Pts',(-16.6200900117121,19.3692101175599,
-6.70211916104053));
#108342=CARTESIAN_POINT('Ctrl Pts',(-16.6147400498285,19.2598264985895,
-6.70800733845812));
#108343=CARTESIAN_POINT('Ctrl Pts',(-16.6191737607425,19.1046963925756,
-6.71645672587226));
#108344=CARTESIAN_POINT('Ctrl Pts',(-16.6219714298163,19.0589291001994,
-6.71896329434194));
#108345=CARTESIAN_POINT('Ctrl Pts',(-16.628356127554,18.9908630336243,-6.72275443083819));
#108346=CARTESIAN_POINT('Ctrl Pts',(-16.6308175885516,18.968471453882,-6.72401191825206));
#108347=CARTESIAN_POINT('Ctrl Pts',(-16.6343250878182,18.9406583429107,
-6.72559123515573));
#108348=CARTESIAN_POINT('Ctrl Pts',(-16.6350356851202,18.9351954453078,
-6.72590227249363));
#108349=CARTESIAN_POINT('Ctrl Pts',(-16.6419010499118,18.8839798565246,
-6.72882665627511));
#108350=CARTESIAN_POINT('Ctrl Pts',(-16.6495290524978,18.8384407793363,
-6.73148942284214));
#108351=CARTESIAN_POINT('Ctrl Pts',(-16.6601486761626,18.7856904313191,
-6.73468473442779));
#108352=CARTESIAN_POINT('Ctrl Pts',(-16.6616993583049,18.7781979794171,
-6.73514121618079));
#108353=CARTESIAN_POINT('Ctrl Pts',(-16.6642506545308,18.7661989701166,
-6.73587672601004));
#108354=CARTESIAN_POINT('Ctrl Pts',(-16.6652254690867,18.7616869147515,
-6.73615431852071));
#108355=CARTESIAN_POINT('Ctrl Pts',(-16.6669833785169,18.7536772110023,
-6.73664895645544));
#108356=CARTESIAN_POINT('Ctrl Pts',(-16.667760607178,18.7501783227761,-6.73686566370459));
#108357=CARTESIAN_POINT('Ctrl Pts',(-16.6694328948811,18.7427393963541,
-6.73732777068667));
#108358=CARTESIAN_POINT('Ctrl Pts',(-16.6703303348727,18.7388000031049,
-6.73757329967693));
#108359=CARTESIAN_POINT('Ctrl Pts',(-16.6727967116562,18.7281149516898,
-6.73824142612402));
#108360=CARTESIAN_POINT('Ctrl Pts',(-16.6743874667519,18.7213744537036,
-6.73866524702791));
#108361=CARTESIAN_POINT('Ctrl Pts',(-16.682637001227,18.687170413667,-6.7408273809394));
#108362=CARTESIAN_POINT('Ctrl Pts',(-16.6898117975037,18.6598357774309,
-6.74259296999075));
#108363=CARTESIAN_POINT('Ctrl Pts',(-16.712457274106,18.5800965700325,-6.74783830432024));
#108364=CARTESIAN_POINT('Ctrl Pts',(-16.7294115317018,18.528139554758,-6.75137725606256));
#108365=CARTESIAN_POINT('Ctrl Pts',(-16.7969219262492,18.3455326422181,
-6.76412363157466));
#108366=CARTESIAN_POINT('Ctrl Pts',(-16.8584109970873,18.2192963971882,
-6.77348418486953));
#108367=CARTESIAN_POINT('Ctrl Pts',(-16.9794541901585,18.0229497807339,
-6.78837879912124));
#108368=CARTESIAN_POINT('Ctrl Pts',(-17.0318942637748,17.9489642843847,
-6.79408884258619));
#108369=CARTESIAN_POINT('Ctrl Pts',(-17.0975627644199,17.8678876773667,
-6.80045486775424));
#108370=CARTESIAN_POINT('Ctrl Pts',(-17.1063087585728,17.857301815866,-6.80128847572375));
#108371=CARTESIAN_POINT('Ctrl Pts',(-17.1205003442702,17.840461197254,-6.80261874543974));
#108372=CARTESIAN_POINT('Ctrl Pts',(-17.125880658652,17.8341521740186,-6.80311805040682));
#108373=CARTESIAN_POINT('Ctrl Pts',(-17.1354996762285,17.823006097242,-6.80400191373796));
#108374=CARTESIAN_POINT('Ctrl Pts',(-17.139723591022,17.8181564723982,-6.80438707506775));
#108375=CARTESIAN_POINT('Ctrl Pts',(-17.1485704758822,17.8080920243343,
-6.80518768537809));
#108376=CARTESIAN_POINT('Ctrl Pts',(-17.1531972341162,17.8028806225004,
-6.80560296985693));
#108377=CARTESIAN_POINT('Ctrl Pts',(-17.1652798908828,17.7894057926614,
-6.80667870921732));
#108378=CARTESIAN_POINT('Ctrl Pts',(-17.1727754322762,17.781178078439,-6.80733748840182));
#108379=CARTESIAN_POINT('Ctrl Pts',(-17.2056108239345,17.7457013580921,
-6.81018703159708));
#108380=CARTESIAN_POINT('Ctrl Pts',(-17.2316026522373,17.7190629900207,
-6.8123497891572));
#108381=CARTESIAN_POINT('Ctrl Pts',(-17.3025205197055,17.6501150062675,
-6.81802622880685));
#108382=CARTESIAN_POINT('Ctrl Pts',(-17.3486175935594,17.6090599543998,
-6.82148893816861));
#108383=CARTESIAN_POINT('Ctrl Pts',(-17.510474011078,17.4771271710602,-6.83304165867512));
#108384=CARTESIAN_POINT('Ctrl Pts',(-17.6338736056185,17.3963238434515,
-6.84084414466426));
#108385=CARTESIAN_POINT('Ctrl Pts',(-17.8276038252418,17.2965418731574,
-6.85294326235159));
#108386=CARTESIAN_POINT('Ctrl Pts',(-17.8921409447088,17.2672986072854,
-6.85695772225955));
#108387=CARTESIAN_POINT('Ctrl Pts',(-17.9667339813452,17.2379111281438,
-6.86171041364105));
#108388=CARTESIAN_POINT('Ctrl Pts',(-17.9754764715837,17.2345337369055,
-6.86226915901613));
#108389=CARTESIAN_POINT('Ctrl Pts',(-17.9885018949849,17.2296009146905,
-6.86310458630137));
#108390=CARTESIAN_POINT('Ctrl Pts',(-17.9927680260369,17.2280010288126,
-6.8633786768183));
#108391=CARTESIAN_POINT('Ctrl Pts',(-18.000385584567,17.2251723056559,-6.86386898060121));
#108392=CARTESIAN_POINT('Ctrl Pts',(-18.0037349863966,17.2239381610488,
-6.86408487314373));
#108393=CARTESIAN_POINT('Ctrl Pts',(-18.0109633788425,17.2212954806104,
-6.86455147327139));
#108394=CARTESIAN_POINT('Ctrl Pts',(-18.0148433157067,17.2198898340928,
-6.86480234262199));
#108395=CARTESIAN_POINT('Ctrl Pts',(-18.0256142362982,17.2160232703419,
-6.86549987114949));
#108396=CARTESIAN_POINT('Ctrl Pts',(-18.032513829831,17.2135867499298,-6.86594793840112));
#108397=CARTESIAN_POINT('Ctrl Pts',(-18.0712295120077,17.2001400417858,
-6.86846859594852));
#108398=CARTESIAN_POINT('Ctrl Pts',(-18.103290183334,17.1898549477508,-6.87058013347566));
#108399=CARTESIAN_POINT('Ctrl Pts',(-18.2043692895027,17.1600677288264,
-6.87728319908461));
#108400=CARTESIAN_POINT('Ctrl Pts',(-18.2741394099589,17.1433059507845,
-6.88197474973276));
#108401=CARTESIAN_POINT('Ctrl Pts',(-18.3753408009632,17.124368888511,-6.88876052556498));
#108402=CARTESIAN_POINT('Ctrl Pts',(-18.4061850192679,17.1193013758637,
-6.89082642451158));
#108403=CARTESIAN_POINT('Ctrl Pts',(-18.5985933373778,17.0920503959333,
-6.90366803488408));
#108404=CARTESIAN_POINT('Ctrl Pts',(-18.7621881789397,17.0879110161657,
-6.91432574939461));
#108405=CARTESIAN_POINT('Ctrl Pts',(-18.9482508918191,17.1047363139869,
-6.92583284203347));
#108406=CARTESIAN_POINT('Ctrl Pts',(-18.9718066771048,17.1072656499619,
-6.92727960971582));
#108407=CARTESIAN_POINT('Ctrl Pts',(-19.0049038406595,17.1113825439887,
-6.92929897342414));
#108408=CARTESIAN_POINT('Ctrl Pts',(-19.014483703288,17.112640819711,-6.92988188640347));
#108409=CARTESIAN_POINT('Ctrl Pts',(-19.0299862142399,17.1147850738926,
-6.93082269485222));
#108410=CARTESIAN_POINT('Ctrl Pts',(-19.0359142258081,17.1156306633781,
-6.93118186156488));
#108411=CARTESIAN_POINT('Ctrl Pts',(-19.0482764447246,17.1174475986493,
-6.93192966384728));
#108412=CARTESIAN_POINT('Ctrl Pts',(-19.054709929736,17.1184234820832,-6.93231815158711));
#108413=CARTESIAN_POINT('Ctrl Pts',(-19.0699338547895,17.1208046289212,
-6.93323588982979));
#108414=CARTESIAN_POINT('Ctrl Pts',(-19.0787201767533,17.1222357127958,
-6.93376431632037));
#108415=CARTESIAN_POINT('Ctrl Pts',(-19.1079652454826,17.1271886008144,
-6.93551924328855));
#108416=CARTESIAN_POINT('Ctrl Pts',(-19.1283815922944,17.1309559723268,
-6.9367379476779));
#108417=CARTESIAN_POINT('Ctrl Pts',(-19.2371590455703,17.1526875904462,
-6.94320143754973));
#108418=CARTESIAN_POINT('Ctrl Pts',(-19.3243649225639,17.1759837954818,
-6.94827249001944));
#108419=CARTESIAN_POINT('Ctrl Pts',(-19.5349343910049,17.246917277589,-6.96052633409362));
#108420=CARTESIAN_POINT('Ctrl Pts',(-19.6558194708651,17.3006691694042,
-6.96756063895633));
#108421=CARTESIAN_POINT('Ctrl Pts',(-19.8394367948869,17.4038262746204,
-6.97919951131585));
#108422=CARTESIAN_POINT('Ctrl Pts',(-19.9057603173634,17.4461084208513,
-6.98363193070267));
#108423=CARTESIAN_POINT('Ctrl Pts',(-19.9773035017372,17.4975309849909,
-6.98885340915815));
#108424=CARTESIAN_POINT('Ctrl Pts',(-19.984997480935,17.5031402405748,-6.98942094753584));
#108425=CARTESIAN_POINT('Ctrl Pts',(-19.9963403970242,17.511527508061,-6.99026700976626));
#108426=CARTESIAN_POINT('Ctrl Pts',(-20.0000186902265,17.5142658711791,
-6.99054284508725));
#108427=CARTESIAN_POINT('Ctrl Pts',(-20.0064228817851,17.5190659908539,
-6.99102572912091));
#108428=CARTESIAN_POINT('Ctrl Pts',(-20.0091527195476,17.5211224236487,
-6.9912324042085));
#108429=CARTESIAN_POINT('Ctrl Pts',(-20.0150418834089,17.525581225576,-6.99168010982486));
#108430=CARTESIAN_POINT('Ctrl Pts',(-20.0181993896464,17.5279858350976,
-6.99192129442607));
#108431=CARTESIAN_POINT('Ctrl Pts',(-20.0265812281815,17.5344063729837,
-6.99256454690003));
#108432=CARTESIAN_POINT('Ctrl Pts',(-20.0317935544019,17.5384378011236,
-6.99296768502342));
#108433=CARTESIAN_POINT('Ctrl Pts',(-20.0433747956963,17.5474819403293,
-6.99387024860555));
#108434=CARTESIAN_POINT('Ctrl Pts',(-20.0497338839925,17.5525069996192,
-6.9943704856369));
#108435=CARTESIAN_POINT('Ctrl Pts',(-20.0689204842056,17.5678483719936,
-6.9958935592754));
#108436=CARTESIAN_POINT('Ctrl Pts',(-20.0816563706499,17.578277658892,-6.99692337480648));
#108437=CARTESIAN_POINT('Ctrl Pts',(-20.1287027893391,17.6177289679715,
-7.00079427755288));
#108438=CARTESIAN_POINT('Ctrl Pts',(-20.1622064138246,17.6476912088858,
-7.00368541326625));
#108439=CARTESIAN_POINT('Ctrl Pts',(-20.248824004471,17.7302627623181,-7.01147319279298));
#108440=CARTESIAN_POINT('Ctrl Pts',(-20.3001487515164,17.7846578152127,
-7.01642138706372));
#108441=CARTESIAN_POINT('Ctrl Pts',(-20.4495444043509,17.9607981133953,
-7.031679511117));
#108442=CARTESIAN_POINT('Ctrl Pts',(-20.5371182239641,18.0907862353464,
-7.04186364993614));
#108443=CARTESIAN_POINT('Ctrl Pts',(-20.6206850155805,18.250437389378,-7.05296529491066));
#108444=CARTESIAN_POINT('Ctrl Pts',(-20.6314155510558,18.2718114262032,
-7.05442602382381));
#108445=CARTESIAN_POINT('Ctrl Pts',(-20.6459864025894,18.3021044725683,
-7.05646143602513));
#108446=CARTESIAN_POINT('Ctrl Pts',(-20.6501307560522,18.3108744453788,
-7.05704665600075));
#108447=CARTESIAN_POINT('Ctrl Pts',(-20.656738795033,18.3251103539889,-7.0579901865129));
#108448=CARTESIAN_POINT('Ctrl Pts',(-20.6592397583875,18.3305587397744,
-7.05834978263468));
#108449=CARTESIAN_POINT('Ctrl Pts',(-20.6644047567989,18.3419380081105,
-7.05909770203643));
#108450=CARTESIAN_POINT('Ctrl Pts',(-20.667064684467,18.3478706945424,-7.0594858808922));
#108451=CARTESIAN_POINT('Ctrl Pts',(-20.673289288512,18.361927120322,-7.06040150549724));
#108452=CARTESIAN_POINT('Ctrl Pts',(-20.6768303331593,18.3700612390023,
-7.06092813776373));
#108453=CARTESIAN_POINT('Ctrl Pts',(-20.6884167855165,18.3971402726274,
-7.0626708696102));
#108454=CARTESIAN_POINT('Ctrl Pts',(-20.6962371957432,18.4161806123037,
-7.06387932326408));
#108455=CARTESIAN_POINT('Ctrl Pts',(-20.7102536332852,18.4517748357084,
-7.06610874928887));
#108456=CARTESIAN_POINT('Ctrl Pts',(-20.7165212951111,18.4682952089492,
-7.06713179939855));
#108457=CARTESIAN_POINT('Ctrl Pts',(-20.7225806056755,18.4848896952038,
-7.06814847058112));
#108458=CARTESIAN_POINT('Ctrl Pts',(-20.7225806151895,18.4848897212595,
-6.84500607926505));
#108459=CARTESIAN_POINT('Ctrl Pts',(-20.7143220134754,18.4622720889823,
-6.84341670129537));
#108460=CARTESIAN_POINT('Ctrl Pts',(-20.7056776513276,18.4397956571551,
-6.84182493616512));
#108461=CARTESIAN_POINT('Ctrl Pts',(-20.6822899809051,18.3819505148498,
-6.83770208830836));
#108462=CARTESIAN_POINT('Ctrl Pts',(-20.6669669998539,18.346826663267,-6.83517292694144));
#108463=CARTESIAN_POINT('Ctrl Pts',(-20.6103477411035,18.2260939710641,
-6.8264140542921));
#108464=CARTESIAN_POINT('Ctrl Pts',(-20.5642446745063,18.1428573145741,
-6.82026493568266));
#108465=CARTESIAN_POINT('Ctrl Pts',(-20.4876289407121,18.0241504991971,
-6.81139913780444));
#108466=CARTESIAN_POINT('Ctrl Pts',(-20.4612924311316,17.986137729419,-6.80854276315538));
#108467=CARTESIAN_POINT('Ctrl Pts',(-20.4265842496443,17.9393902837932,
-6.80500504977845));
#108468=CARTESIAN_POINT('Ctrl Pts',(-20.4193562226583,17.9298258804877,
-6.80427984972165));
#108469=CARTESIAN_POINT('Ctrl Pts',(-20.4076826075114,17.9146486664867,
-6.80312668118412));
#108470=CARTESIAN_POINT('Ctrl Pts',(-20.4032891942628,17.9089962217928,
-6.80269666963867));
#108471=CARTESIAN_POINT('Ctrl Pts',(-20.3949230794441,17.8983445631575,
-6.80188527536604));
#108472=CARTESIAN_POINT('Ctrl Pts',(-20.3909562767742,17.8933408369608,
-6.80150366454686));
#108473=CARTESIAN_POINT('Ctrl Pts',(-20.381926168831,17.8820555183535,-6.80064192087892));
#108474=CARTESIAN_POINT('Ctrl Pts',(-20.3768494522396,17.8757847464745,
-6.80016233273327));
#108475=CARTESIAN_POINT('Ctrl Pts',(-20.3617613994614,17.8573642803901,
-6.79875117671033));
#108476=CARTESIAN_POINT('Ctrl Pts',(-20.351650110109,17.845296893096,-6.79782366284704));
#108477=CARTESIAN_POINT('Ctrl Pts',(-20.2603461998441,17.738766476022,-6.78960486120131));
#108478=CARTESIAN_POINT('Ctrl Pts',(-20.1710943863378,17.6515225211304,
-6.7826764506399));
#108479=CARTESIAN_POINT('Ctrl Pts',(-19.9449994152531,17.4665098406586,
-6.76672098599696));
#108480=CARTESIAN_POINT('Ctrl Pts',(-19.8032014748065,17.3761816864413,
-6.75786105594184));
#108481=CARTESIAN_POINT('Ctrl Pts',(-19.6328583142164,17.2941779716061,
-6.74686290809761));
#108482=CARTESIAN_POINT('Ctrl Pts',(-19.6133098192053,17.2851321129742,
-6.74559528639951));
#108483=CARTESIAN_POINT('Ctrl Pts',(-19.5878774508088,17.273831475815,-6.7439348128286));
#108484=CARTESIAN_POINT('Ctrl Pts',(-19.5821160421196,17.271302144944,-6.74355790950506));
#108485=CARTESIAN_POINT('Ctrl Pts',(-19.5732581848009,17.2674604431169,
-6.7429771770025));
#108486=CARTESIAN_POINT('Ctrl Pts',(-19.5701696836641,17.2661296779264,
-6.74277445606564));
#108487=CARTESIAN_POINT('Ctrl Pts',(-19.5637959026683,17.2634013487738,
-6.74235558845871));
#108488=CARTESIAN_POINT('Ctrl Pts',(-19.5605102829406,17.2620047465699,
-6.7421393841452));
#108489=CARTESIAN_POINT('Ctrl Pts',(-19.5530175758088,17.2588422121783,
-6.74164570564581));
#108490=CARTESIAN_POINT('Ctrl Pts',(-19.5488083187603,17.2570815726303,
-6.74136791603673));
#108491=CARTESIAN_POINT('Ctrl Pts',(-19.5378428223199,17.2525365418416,
-6.7406431409666));
#108492=CARTESIAN_POINT('Ctrl Pts',(-19.5310778652378,17.2497735283403,
-6.74019491368503));
#108493=CARTESIAN_POINT('Ctrl Pts',(-19.4877772395379,17.2323492767911,
-6.73731960983018));
#108494=CARTESIAN_POINT('Ctrl Pts',(-19.4508553833683,17.2186755495305,
-6.73483929506114));
#108495=CARTESIAN_POINT('Ctrl Pts',(-19.2328008268541,17.1447664450555,
-6.72011176022653));
#108496=CARTESIAN_POINT('Ctrl Pts',(-19.0445651574952,17.1082199585982,
-6.70718190373954));
#108497=CARTESIAN_POINT('Ctrl Pts',(-18.7989504908739,17.0942792503341,
-6.6913689942318));
#108498=CARTESIAN_POINT('Ctrl Pts',(-18.7438321414033,17.0933056291223,
-6.68787969213037));
#108499=CARTESIAN_POINT('Ctrl Pts',(-18.6544382366206,17.0952174711428,
-6.68232189017504));
#108500=CARTESIAN_POINT('Ctrl Pts',(-18.62016323703,17.0967844974204,-6.68021494757116));
#108501=CARTESIAN_POINT('Ctrl Pts',(-18.5751577141615,17.0999398508508,
-6.67747833512118));
#108502=CARTESIAN_POINT('Ctrl Pts',(-18.5643814100127,17.1007783609742,
-6.67682532216682));
#108503=CARTESIAN_POINT('Ctrl Pts',(-18.5467388892616,17.1022871557849,
-6.67575981217204));
#108504=CARTESIAN_POINT('Ctrl Pts',(-18.5398687887741,17.1029085272378,
-6.67534578563145));
#108505=CARTESIAN_POINT('Ctrl Pts',(-18.5265742260694,17.1041765053469,
-6.67454626925512));
#108506=CARTESIAN_POINT('Ctrl Pts',(-18.5201494520033,17.1048189456127,
-6.67416065306325));
#108507=CARTESIAN_POINT('Ctrl Pts',(-18.5053189933518,17.1063704656718,
-6.67327223785971));
#108508=CARTESIAN_POINT('Ctrl Pts',(-18.4969155784984,17.1073005300631,
-6.67277010488811));
#108509=CARTESIAN_POINT('Ctrl Pts',(-18.4743247514978,17.1099378982511,
-6.67142351508182));
#108510=CARTESIAN_POINT('Ctrl Pts',(-18.4601485262874,17.1117385643171,
-6.67058199951463));
#108511=CARTESIAN_POINT('Ctrl Pts',(-18.3302621524138,17.1295748725372,
-6.66290141150551));
#108512=CARTESIAN_POINT('Ctrl Pts',(-18.2160397733325,17.1550191451251,
-6.65637889965437));
#108513=CARTESIAN_POINT('Ctrl Pts',(-17.9491280413759,17.2381485870596,
-6.64107455735116));
#108514=CARTESIAN_POINT('Ctrl Pts',(-17.7998848724256,17.3042793139915,
-6.63247574464883));
#108515=CARTESIAN_POINT('Ctrl Pts',(-17.6316679018545,17.4033463694684,
-6.62126682880853));
#108516=CARTESIAN_POINT('Ctrl Pts',(-17.6040170937382,17.4205011666582,
-6.619369121449));
#108517=CARTESIAN_POINT('Ctrl Pts',(-17.57071039928,17.442243729078,-6.61700087346868));
#108518=CARTESIAN_POINT('Ctrl Pts',(-17.564666925745,17.4462332734673,-6.61656776808855));
#108519=CARTESIAN_POINT('Ctrl Pts',(-17.5552256638617,17.4525356251233,
-6.61588563279881));
#108520=CARTESIAN_POINT('Ctrl Pts',(-17.5518138742039,17.4548274980619,
-6.61563798963811));
#108521=CARTESIAN_POINT('Ctrl Pts',(-17.5454496171984,17.4591296435288,
-6.61517386531391));
#108522=CARTESIAN_POINT('Ctrl Pts',(-17.542495555898,17.4611374575784,-6.61495754968225));
#108523=CARTESIAN_POINT('Ctrl Pts',(-17.5357645335208,17.4657373403748,
-6.61446264424152));
#108524=CARTESIAN_POINT('Ctrl Pts',(-17.5319909088529,17.4683341892092,
-6.6141837327842));
#108525=CARTESIAN_POINT('Ctrl Pts',(-17.5204198562389,17.476352362637,-6.61332411128808));
#108526=CARTESIAN_POINT('Ctrl Pts',(-17.5126505815199,17.4818138384214,
-6.61274076420295));
#108527=CARTESIAN_POINT('Ctrl Pts',(-17.4068825182073,17.5572327798541,
-6.60471755657163));
#108528=CARTESIAN_POINT('Ctrl Pts',(-17.3150002233062,17.6353668714839,
-6.59679439738272));
#108529=CARTESIAN_POINT('Ctrl Pts',(-17.1537485064117,17.7980910068835,
-6.58165946836446));
#108530=CARTESIAN_POINT('Ctrl Pts',(-17.0832853054485,17.8810935801749,
-6.5744754061784));
#108531=CARTESIAN_POINT('Ctrl Pts',(-16.9757264633497,18.0295885239447,
-6.56269744811341));
#108532=CARTESIAN_POINT('Ctrl Pts',(-16.9351698668512,18.0923082771127,
-6.55800287880983));
#108533=CARTESIAN_POINT('Ctrl Pts',(-16.8886708917684,18.1733096987392,
-6.55228154797359));
#108534=CARTESIAN_POINT('Ctrl Pts',(-16.8795508992046,18.1896972794019,
-6.55114057520357));
#108535=CARTESIAN_POINT('Ctrl Pts',(-16.8665942314234,18.2137248621869,
-6.54949110757985));
#108536=CARTESIAN_POINT('Ctrl Pts',(-16.8625843571402,18.2212699863012,
-6.54897645862849));
#108537=CARTESIAN_POINT('Ctrl Pts',(-16.8556288987312,18.2345510365307,
-6.54807629759175));
#108538=CARTESIAN_POINT('Ctrl Pts',(-16.8526636557792,18.2402764895799,
-6.54769009297099));
#108539=CARTESIAN_POINT('Ctrl Pts',(-16.8469529201325,18.2514275476424,
-6.54694146807916));
#108540=CARTESIAN_POINT('Ctrl Pts',(-16.8442045577679,18.256851604484,-6.54657894953628));
#108541=CARTESIAN_POINT('Ctrl Pts',(-16.8376844453821,18.2698581216867,
-6.54571349320474));
#108542=CARTESIAN_POINT('Ctrl Pts',(-16.8339347305135,18.277451558483,-6.54521132939325));
#108543=CARTESIAN_POINT('Ctrl Pts',(-16.820534356187,18.3050034790034,-6.54340029987387));
#108544=CARTESIAN_POINT('Ctrl Pts',(-16.8111515678527,18.32509118537,-6.54210072537341));
#108545=CARTESIAN_POINT('Ctrl Pts',(-16.7264458176462,18.5141273633586,
-6.53005381234589));
#108546=CARTESIAN_POINT('Ctrl Pts',(-16.6732559435664,18.692111505969,-6.52015640957286));
#108547=CARTESIAN_POINT('Ctrl Pts',(-16.6310807936875,18.9542764684892,
-6.50568281724552));
#108548=CARTESIAN_POINT('Ctrl Pts',(-16.6228376561477,19.0344562683373,
-6.50125469187608));
#108549=CARTESIAN_POINT('Ctrl Pts',(-16.6175417613026,19.1510043347839,
-6.49458190957017));
#108550=CARTESIAN_POINT('Ctrl Pts',(-16.6168261179675,19.1871387822826,
-6.4924800688684));
#108551=CARTESIAN_POINT('Ctrl Pts',(-16.6170788824418,19.2307439697001,
-6.48988507322991));
#108552=CARTESIAN_POINT('Ctrl Pts',(-16.6171617641848,19.2382162068831,
-6.48943831376105));
#108553=CARTESIAN_POINT('Ctrl Pts',(-16.6173523789404,19.2498479094962,
-6.4887394121124));
#108554=CARTESIAN_POINT('Ctrl Pts',(-16.6174328179095,19.2540078460606,
-6.48848877116767));
#108555=CARTESIAN_POINT('Ctrl Pts',(-16.6176049653505,19.2617323563995,
-6.48802203975642));
#108556=CARTESIAN_POINT('Ctrl Pts',(-16.6176934163981,19.2652969453461,
-6.48780613339093));
#108557=CARTESIAN_POINT('Ctrl Pts',(-16.617914101094,19.2733682300484,-6.48731607123002));
#108558=CARTESIAN_POINT('Ctrl Pts',(-16.618051725722,19.2778747140442,-6.48704161856702));
#108559=CARTESIAN_POINT('Ctrl Pts',(-16.6185017589033,19.2912141579863,
-6.48622682442084));
#108560=CARTESIAN_POINT('Ctrl Pts',(-16.618855085394,19.3000455119049,-6.48568427695643));
#108561=CARTESIAN_POINT('Ctrl Pts',(-16.6218723043404,19.3652375790354,
-6.48165753514319));
#108562=CARTESIAN_POINT('Ctrl Pts',(-16.6267329986812,19.4214690410508,
-6.47806481547717));
#108563=CARTESIAN_POINT('Ctrl Pts',(-16.654862484207,19.6432002214296,-6.46359157221598));
#108564=CARTESIAN_POINT('Ctrl Pts',(-16.6954432956854,19.8058983258611,
-6.45234682466899));
#108565=CARTESIAN_POINT('Ctrl Pts',(-16.7754971229906,20.0168400066529,
-6.43780560662173));
#108566=CARTESIAN_POINT('Ctrl Pts',(-16.7985146582946,20.0706563838884,
-6.43409242974263));
#108567=CARTESIAN_POINT('Ctrl Pts',(-16.8391736067629,20.1557778306183,
-6.42822140406911));
#108568=CARTESIAN_POINT('Ctrl Pts',(-16.8554319310722,20.1877059261988,
-6.4260194916168));
#108569=CARTESIAN_POINT('Ctrl Pts',(-16.8777223982199,20.2288619811032,
-6.42317971533229));
#108570=CARTESIAN_POINT('Ctrl Pts',(-16.8830263732737,20.2384756385058,
-6.42251625139232));
#108571=CARTESIAN_POINT('Ctrl Pts',(-16.8918025091519,20.2540941987987,
-6.4214380561763));
#108572=CARTESIAN_POINT('Ctrl Pts',(-16.8952297634089,20.2601239782134,
-6.42102172455256));
#108573=CARTESIAN_POINT('Ctrl Pts',(-16.9018975938012,20.2717220549832,
-6.42022073097131));
#108574=CARTESIAN_POINT('Ctrl Pts',(-16.9051340726756,20.2772926080656,
-6.41983592702379));
#108575=CARTESIAN_POINT('Ctrl Pts',(-16.91263135217,20.29006219788,-6.41895358075498));
#108576=CARTESIAN_POINT('Ctrl Pts',(-16.9169095128342,20.297250957518,-6.41845667524244));
#108577=CARTESIAN_POINT('Ctrl Pts',(-16.9284521998043,20.3163875602612,
-6.41713329240401));
#108578=CARTESIAN_POINT('Ctrl Pts',(-16.9357927533133,20.3282892325262,
-6.41630959801596));
#108579=CARTESIAN_POINT('Ctrl Pts',(-16.9968745760143,20.4251633150974,
-6.40959772715613));
#108580=CARTESIAN_POINT('Ctrl Pts',(-17.0564919467087,20.5062867489956,
-6.40393904103445));
#108581=CARTESIAN_POINT('Ctrl Pts',(-17.2327398687421,20.7134283558584,
-6.38895543931456));
#108582=CARTESIAN_POINT('Ctrl Pts',(-17.3592547165705,20.8299925173283,
-6.37994389051388));
#108583=CARTESIAN_POINT('Ctrl Pts',(-17.5308108760238,20.9533019762175,
-6.36790651871291));
#108584=CARTESIAN_POINT('Ctrl Pts',(-17.5638514432103,20.975662045985,-6.36559298713685));
#108585=CARTESIAN_POINT('Ctrl Pts',(-17.6039858000269,21.0011999835059,
-6.36276336840678));
#108586=CARTESIAN_POINT('Ctrl Pts',(-17.6104925632376,21.0052906978873,
-6.36230402440016));
#108587=CARTESIAN_POINT('Ctrl Pts',(-17.6205951005058,21.0115655302254,
-6.36158968850719));
#108588=CARTESIAN_POINT('Ctrl Pts',(-17.624175429748,21.0137745620049,-6.36133630688304));
#108589=CARTESIAN_POINT('Ctrl Pts',(-17.630799218448,21.0178341714007,-6.36086708381862));
#108590=CARTESIAN_POINT('Ctrl Pts',(-17.6338407731781,21.0196877459752,
-6.36065144311388));
#108591=CARTESIAN_POINT('Ctrl Pts',(-17.640691805315,21.0238392051238,-6.36016531637365));
#108592=CARTESIAN_POINT('Ctrl Pts',(-17.6445038316379,21.0261327473458,
-6.35989455408282));
#108593=CARTESIAN_POINT('Ctrl Pts',(-17.6542761337772,21.0319704717892,
-6.35919980170283));
#108594=CARTESIAN_POINT('Ctrl Pts',(-17.6602465925175,21.0354973837458,
-6.35877473024137));
#108595=CARTESIAN_POINT('Ctrl Pts',(-17.6952237161171,21.0559281728967,
-6.35628146000999));
#108596=CARTESIAN_POINT('Ctrl Pts',(-17.7246101391587,21.0721684361755,
-6.35417456947352));
#108597=CARTESIAN_POINT('Ctrl Pts',(-17.770557674362,21.0961528847494,-6.35087603535773));
#108598=CARTESIAN_POINT('Ctrl Pts',(-17.7868553396699,21.1043936384059,
-6.34970522002475));
#108599=CARTESIAN_POINT('Ctrl Pts',(-17.8254409867647,21.1232812451234,
-6.34693460951328));
#108600=CARTESIAN_POINT('Ctrl Pts',(-17.8478126038333,21.1337508609787,
-6.34532929755426));
#108601=CARTESIAN_POINT('Ctrl Pts',(-17.9113735152393,21.1621515713041,
-6.34078043255332));
#108602=CARTESIAN_POINT('Ctrl Pts',(-17.9529573742445,21.1791664119522,
-6.33781864804257));
#108603=CARTESIAN_POINT('Ctrl Pts',(-18.0975169317308,21.2330124952325,
-6.32762842442968));
#108604=CARTESIAN_POINT('Ctrl Pts',(-18.2027949927039,21.2631866226279,
-6.32039839227555));
#108605=CARTESIAN_POINT('Ctrl Pts',(-18.3638784422062,21.2961211313912,
-6.30983055555864));
#108606=CARTESIAN_POINT('Ctrl Pts',(-18.4182309585997,21.3050417454674,
-6.30634435451977));
#108607=CARTESIAN_POINT('Ctrl Pts',(-18.5068944692338,21.3160623261965,
-6.3007909136273));
#108608=CARTESIAN_POINT('Ctrl Pts',(-18.5410147437896,21.3194641865828,
-6.29868530619467));
#108609=CARTESIAN_POINT('Ctrl Pts',(-18.5859799012722,21.3228465432972,
-6.29595014797637));
#108610=CARTESIAN_POINT('Ctrl Pts',(-18.5967617714073,21.3235746016313,
-6.29529728509838));
#108611=CARTESIAN_POINT('Ctrl Pts',(-18.6144340882067,21.3246320796817,
-6.29423195721404));
#108612=CARTESIAN_POINT('Ctrl Pts',(-18.6213213086204,21.3250104280214,
-6.29381796371635));
#108613=CARTESIAN_POINT('Ctrl Pts',(-18.6346591958927,21.3256777761072,
-6.29301846778467));
#108614=CARTESIAN_POINT('Ctrl Pts',(-18.6411095693651,21.325970936312,-6.29263283922168));
#108615=CARTESIAN_POINT('Ctrl Pts',(-18.6560100725481,21.326579843261,-6.29174433354024));
#108616=CARTESIAN_POINT('Ctrl Pts',(-18.6644609907015,21.3268744838357,
-6.29124212289746));
#108617=CARTESIAN_POINT('Ctrl Pts',(-18.68720167596,21.3275309442009,-6.28989518723335));
#108618=CARTESIAN_POINT('Ctrl Pts',(-18.7014938729718,21.3277986884734,
-6.2890534058719));
#108619=CARTESIAN_POINT('Ctrl Pts',(-18.8329520787702,21.328929634035,-6.28135190565202));
#108620=CARTESIAN_POINT('Ctrl Pts',(-18.9500047707518,21.3202094924316,
-6.27481081589188));
#108621=CARTESIAN_POINT('Ctrl Pts',(-19.227594783444,21.2761651349409,-6.25942589144886));
#108622=CARTESIAN_POINT('Ctrl Pts',(-19.3858920386363,21.2317838238735,
-6.25076847213039));
#108623=CARTESIAN_POINT('Ctrl Pts',(-19.5663317561777,21.1577630041048,
-6.23955367023813));
#108624=CARTESIAN_POINT('Ctrl Pts',(-19.5949289670148,21.1452862837592,
-6.23773215292194));
#108625=CARTESIAN_POINT('Ctrl Pts',(-19.6297251086953,21.129180550204,-6.2354487192003));
#108626=CARTESIAN_POINT('Ctrl Pts',(-19.6361965599818,21.126145283619,-6.23502114721715));
#108627=CARTESIAN_POINT('Ctrl Pts',(-19.646346070374,21.1213220597708,-6.2343458117799));
#108628=CARTESIAN_POINT('Ctrl Pts',(-19.6500346006386,21.1195560861436,
-6.23409938980113));
#108629=CARTESIAN_POINT('Ctrl Pts',(-19.6569379777609,21.1162263041503,
-6.23363628738182));
#108630=CARTESIAN_POINT('Ctrl Pts',(-19.6601539882115,21.1146650362561,
-6.23341976477569));
#108631=CARTESIAN_POINT('Ctrl Pts',(-19.6675103803381,21.1110706949841,
-6.23292270314923));
#108632=CARTESIAN_POINT('Ctrl Pts',(-19.671648069908,21.1090322368717,-6.23264183161785));
#108633=CARTESIAN_POINT('Ctrl Pts',(-19.6824718198024,21.103655819941,-6.23190377325335));
#108634=CARTESIAN_POINT('Ctrl Pts',(-19.6891468576182,21.1002959858926,
-6.23144527038847));
#108635=CARTESIAN_POINT('Ctrl Pts',(-19.7338277752976,21.0775088511716,
-6.2283544045501));
#108636=CARTESIAN_POINT('Ctrl Pts',(-19.771253658907,21.0569726842075,-6.2256594437529));
#108637=CARTESIAN_POINT('Ctrl Pts',(-19.8142373859244,21.0316669306559,
-6.22246032614407));
#108638=CARTESIAN_POINT('Ctrl Pts',(-19.8204257537986,21.0279810020234,
-6.22199716670866));
#108639=CARTESIAN_POINT('Ctrl Pts',(-19.9612667849399,20.9431162177966,
-6.21139892056264));
#108640=CARTESIAN_POINT('Ctrl Pts',(-20.0864795940046,20.8472189992898,
-6.20082566701259));
#108641=CARTESIAN_POINT('Ctrl Pts',(-20.2683631239063,20.6726489957371,
-6.18444653877917));
#108642=CARTESIAN_POINT('Ctrl Pts',(-20.3323175750643,20.6024284380669,
-6.17842091286517));
#108643=CARTESIAN_POINT('Ctrl Pts',(-20.4046232442814,20.5114468131507,
-6.17128283460061));
#108644=CARTESIAN_POINT('Ctrl Pts',(-20.4176410418737,20.4945485314317,
-6.16998278769079));
#108645=CARTESIAN_POINT('Ctrl Pts',(-20.435785262638,20.4702445777675,-6.16814856148964));
#108646=CARTESIAN_POINT('Ctrl Pts',(-20.4411229320124,20.462998916004,-6.16760612817427));
#108647=CARTESIAN_POINT('Ctrl Pts',(-20.4502504309371,20.4504418205428,
-6.16667354115692));
#108648=CARTESIAN_POINT('Ctrl Pts',(-20.4540621751653,20.4451465404267,
-6.16628254019508));
#108649=CARTESIAN_POINT('Ctrl Pts',(-20.4613129507941,20.4349749073252,
-6.16553576202989));
#108650=CARTESIAN_POINT('Ctrl Pts',(-20.4647559590963,20.4301014785153,
-6.16517983400147));
#108651=CARTESIAN_POINT('Ctrl Pts',(-20.4736538398603,20.4173932423729,
-6.16425649597891));
#108652=CARTESIAN_POINT('Ctrl Pts',(-20.4790764412075,20.4095359221416,
-6.16369032208042));
#108653=CARTESIAN_POINT('Ctrl Pts',(-20.4973780625558,20.3826294352831,
-6.16176726432045));
#108654=CARTESIAN_POINT('Ctrl Pts',(-20.5100000826025,20.3634068260241,
-6.16042007253108));
#108655=CARTESIAN_POINT('Ctrl Pts',(-20.6162011446523,20.1957782924256,
-6.14888912527794));
#108656=CARTESIAN_POINT('Ctrl Pts',(-20.6913089129596,20.0364804387942,
-6.1394558683824));
#108657=CARTESIAN_POINT('Ctrl Pts',(-20.7729859957996,19.7870200369861,
-6.12517356199045));
#108658=CARTESIAN_POINT('Ctrl Pts',(-20.7949379458987,19.7027269166773,
-6.12040921269416));
#108659=CARTESIAN_POINT('Ctrl Pts',(-20.8189001284145,19.5802038973624,
-6.11328134095437));
#108660=CARTESIAN_POINT('Ctrl Pts',(-20.8251640445067,19.542892456784,-6.11108394711787));
#108661=CARTESIAN_POINT('Ctrl Pts',(-20.8314778225086,19.4979374848787,
-6.10838299811422));
#108662=CARTESIAN_POINT('Ctrl Pts',(-20.8324907016688,19.4904335470698,
-6.10793037519611));
#108663=CARTESIAN_POINT('Ctrl Pts',(-20.8340004990705,19.4787767650944,
-6.1072242799401));
#108664=CARTESIAN_POINT('Ctrl Pts',(-20.8345254153759,19.4746275226261,
-6.10697235921564));
#108665=CARTESIAN_POINT('Ctrl Pts',(-20.8354748337342,19.4669398830099,
-6.10650447622598));
#108666=CARTESIAN_POINT('Ctrl Pts',(-20.8359026977808,19.4634019592107,
-6.10628870586585));
#108667=CARTESIAN_POINT('Ctrl Pts',(-20.836848273436,19.4554140124471,-6.1058005355452));
#108668=CARTESIAN_POINT('Ctrl Pts',(-20.8373607907553,19.4509634422841,
-6.10552784856523));
#108669=CARTESIAN_POINT('Ctrl Pts',(-20.8388276186781,19.4378600411612,
-6.10472301637945));
#108670=CARTESIAN_POINT('Ctrl Pts',(-20.8397426748065,19.4292030342257,
-6.10418874306042));
#108671=CARTESIAN_POINT('Ctrl Pts',(-20.8458591846126,19.367711116328,-6.10037684633282));
#108672=CARTESIAN_POINT('Ctrl Pts',(-20.8491244446042,19.3147070409703,
-6.0970030715376));
#108673=CARTESIAN_POINT('Ctrl Pts',(-20.8507874983554,19.2452051698429,
-6.09251070877059));
#108674=CARTESIAN_POINT('Ctrl Pts',(-20.8509892979952,19.2287651387287,
-6.09144303796163));
#108675=CARTESIAN_POINT('Ctrl Pts',(-20.8510113338403,19.1935501678798,
-6.08914730328518));
#108676=CARTESIAN_POINT('Ctrl Pts',(-20.8507733287336,19.1747765698913,
-6.08791808606016));
#108677=CARTESIAN_POINT('Ctrl Pts',(-20.8462294574967,18.9999094588411,
-6.076431256371));
#108678=CARTESIAN_POINT('Ctrl Pts',(-20.8249133169856,18.8447155084867,
-6.06600952224626));
#108679=CARTESIAN_POINT('Ctrl Pts',(-20.7855431282212,18.6886181110422,
-6.05574908623547));
#108680=CARTESIAN_POINT('Ctrl Pts',(-20.7843532949711,18.6839673528277,
-6.05544354651447));
#108681=CARTESIAN_POINT('Ctrl Pts',(-20.7672425722882,18.6180208430043,
-6.05111338419313));
#108682=CARTESIAN_POINT('Ctrl Pts',(-20.7485937396552,18.5574611490693,
-6.04716677887305));
#108683=CARTESIAN_POINT('Ctrl Pts',(-20.7257113393618,18.4935071735124,
-6.04302921523241));
#108684=CARTESIAN_POINT('Ctrl Pts',(-20.7241529735247,18.4891959008834,
-6.0427504354363));
#108685=CARTESIAN_POINT('Ctrl Pts',(-20.7225806138063,18.4848897174713,
-6.04247212253779));
#108686=CARTESIAN_POINT('Origin',(-18.734,19.211,0.));
#108687=CARTESIAN_POINT('',(-20.7225806829213,18.484889906755,-5.2445270986103));
#108688=CARTESIAN_POINT('',(-20.7225806137986,18.4848897174502,-5.46434831804488));
#108689=CARTESIAN_POINT('',(-20.7225806137986,18.4848897174502,0.));
#108690=CARTESIAN_POINT('',(-20.8509993557837,19.2093484518076,-5.51218501636556));
#108691=CARTESIAN_POINT('Ctrl Pts',(-20.7225806137986,18.4848897174502,
-5.46434831804488));
#108692=CARTESIAN_POINT('Ctrl Pts',(-20.7233024841825,18.4868666863565,
-5.46447496720223));
#108693=CARTESIAN_POINT('Ctrl Pts',(-20.7240214029106,18.4888447221103,
-5.46460179002157));
#108694=CARTESIAN_POINT('Ctrl Pts',(-20.7259509440324,18.4941784303195,
-5.46494405560274));
#108695=CARTESIAN_POINT('Ctrl Pts',(-20.7271560109878,18.4975360262837,
-5.46515982705691));
#108696=CARTESIAN_POINT('Ctrl Pts',(-20.7297430820435,18.5048019154282,
-5.4656274508845));
#108697=CARTESIAN_POINT('Ctrl Pts',(-20.7311220758324,18.5087111721524,
-5.46587947189699));
#108698=CARTESIAN_POINT('Ctrl Pts',(-20.7349315291103,18.5196124017892,
-5.46658338460756));
#108699=CARTESIAN_POINT('Ctrl Pts',(-20.7373367833058,18.5266130304581,
-5.46703672596418));
#108700=CARTESIAN_POINT('Ctrl Pts',(-20.7509022232985,18.5667803152235,
-5.46964468032722));
#108701=CARTESIAN_POINT('Ctrl Pts',(-20.7612746976398,18.6002049846049,
-5.47184140961292));
#108702=CARTESIAN_POINT('Ctrl Pts',(-20.7916316012822,18.7073407034207,
-5.47893320443435));
#108703=CARTESIAN_POINT('Ctrl Pts',(-20.8084577951946,18.7818802512658,
-5.48394075702676));
#108704=CARTESIAN_POINT('Ctrl Pts',(-20.8409451160576,18.9735153717483,
-5.49676495883049));
#108705=CARTESIAN_POINT('Ctrl Pts',(-20.8509072796362,19.0913227436705,
-5.50459118708685));
#108706=CARTESIAN_POINT('Ctrl Pts',(-20.8509993557837,19.2093484518076,
-5.51218501636556));
#108707=CARTESIAN_POINT('Ctrl Pts',(-20.8509993578191,19.2093510629101,
-5.51218518436507));
#108708=CARTESIAN_POINT('Ctrl Pts',(-20.8510649772347,19.2935970062879,
-5.51760560536095));
#108709=CARTESIAN_POINT('Ctrl Pts',(-20.8461018019886,19.377781816377,-5.52290050009876));
#108710=CARTESIAN_POINT('Ctrl Pts',(-20.8349011953471,19.4717899931963,
-5.52867288887937));
#108711=CARTESIAN_POINT('Ctrl Pts',(-20.8335940955098,19.4821123260401,
-5.52930486670546));
#108712=CARTESIAN_POINT('Ctrl Pts',(-20.8312616515329,19.4995022658,-5.53036653139996));
#108713=CARTESIAN_POINT('Ctrl Pts',(-20.8302765594365,19.5065750000842,
-5.5307974806336));
#108714=CARTESIAN_POINT('Ctrl Pts',(-20.8283990631231,19.5195732817317,
-5.53158796381311));
#108715=CARTESIAN_POINT('Ctrl Pts',(-20.8275172536352,19.5255002634194,
-5.53194782910823));
#108716=CARTESIAN_POINT('Ctrl Pts',(-20.8256463308097,19.5377188201829,
-5.53268852674375));
#108717=CARTESIAN_POINT('Ctrl Pts',(-20.824653966422,19.5440098417555,-5.53306925197143));
#108718=CARTESIAN_POINT('Ctrl Pts',(-20.8223696977555,19.5580780266519,
-5.53391924827786));
#108719=CARTESIAN_POINT('Ctrl Pts',(-20.8210627052719,19.5658526707286,
-5.53438803530431));
#108720=CARTESIAN_POINT('Ctrl Pts',(-20.8176411998699,19.5855324390729,
-5.53557234197291));
#108721=CARTESIAN_POINT('Ctrl Pts',(-20.8154680491618,19.5974271821816,
-5.53628599504366));
#108722=CARTESIAN_POINT('Ctrl Pts',(-20.8024833895109,19.6652088085229,
-5.54034128987405));
#108723=CARTESIAN_POINT('Ctrl Pts',(-20.7895226757927,19.7206631593222,
-5.54361373169995));
#108724=CARTESIAN_POINT('Ctrl Pts',(-20.7635221396755,19.8146348325442,
-5.54912154478234));
#108725=CARTESIAN_POINT('Ctrl Pts',(-20.7515806173787,19.8534202691554,
-5.55138379417188));
#108726=CARTESIAN_POINT('Ctrl Pts',(-20.7078178717039,19.9822667105859,
-5.55890208225654));
#108727=CARTESIAN_POINT('Ctrl Pts',(-20.6710200248754,20.0705133733609,
-5.56405154180234));
#108728=CARTESIAN_POINT('Ctrl Pts',(-20.5903959124699,20.2321406065725,
-5.57388370684294));
#108729=CARTESIAN_POINT('Ctrl Pts',(-20.5478456863164,20.305940848901,-5.57854916575188));
#108730=CARTESIAN_POINT('Ctrl Pts',(-20.4804070699152,20.4081406417986,
-5.58554356811992));
#108731=CARTESIAN_POINT('Ctrl Pts',(-20.4590211132936,20.4387561417503,
-5.58771340802182));
#108732=CARTESIAN_POINT('Ctrl Pts',(-20.4323561989831,20.47485605703,-5.59038381356568));
#108733=CARTESIAN_POINT('Ctrl Pts',(-20.4278417190277,20.4809000506001,
-5.59083477774178));
#108734=CARTESIAN_POINT('Ctrl Pts',(-20.4207780787938,20.4902521854258,
-5.59153883837267));
#108735=CARTESIAN_POINT('Ctrl Pts',(-20.4182512182753,20.4935772000399,
-5.59179039754004));
#108736=CARTESIAN_POINT('Ctrl Pts',(-20.4135495530391,20.4997261164267,
-5.59225795300536));
#108737=CARTESIAN_POINT('Ctrl Pts',(-20.4113774491847,20.5025520108197,
-5.59247375959621));
#108738=CARTESIAN_POINT('Ctrl Pts',(-20.4064541892731,20.5089237753775,
-5.59296245445069));
#108739=CARTESIAN_POINT('Ctrl Pts',(-20.4036989032278,20.5124663705257,
-5.59323563247517));
#108740=CARTESIAN_POINT('Ctrl Pts',(-20.3955433323692,20.5228838294314,
-5.59404322936797));
#108741=CARTESIAN_POINT('Ctrl Pts',(-20.3901117798278,20.5297339359879,
-5.59457979782281));
#108742=CARTESIAN_POINT('Ctrl Pts',(-20.3510460038105,20.5783805005251,
-5.59842869908015));
#108743=CARTESIAN_POINT('Ctrl Pts',(-20.31587891269,20.6189152196025,-5.60183917827301));
#108744=CARTESIAN_POINT('Ctrl Pts',(-20.2701324030142,20.6677644838475,
-5.60616539159853));
#108745=CARTESIAN_POINT('Ctrl Pts',(-20.2609597733075,20.6773762685511,
-5.60702766373061));
#108746=CARTESIAN_POINT('Ctrl Pts',(-20.1456055252199,20.7959972692869,
-5.61780141355003));
#108747=CARTESIAN_POINT('Ctrl Pts',(-20.0280577798011,20.8933396221013,
-5.62800596734606));
#108748=CARTESIAN_POINT('Ctrl Pts',(-19.8498064431852,21.0111227154827,
-5.64180605232577));
#108749=CARTESIAN_POINT('Ctrl Pts',(-19.7970787269455,21.0427561362285,
-5.64571421651713));
#108750=CARTESIAN_POINT('Ctrl Pts',(-19.7214392817925,21.0837671247593,
-5.65107488895773));
#108751=CARTESIAN_POINT('Ctrl Pts',(-19.6996304608007,21.0951048089231,
-5.65259330477595));
#108752=CARTESIAN_POINT('Ctrl Pts',(-19.661171483041,21.1142551123886,-5.65522440798555));
#108753=CARTESIAN_POINT('Ctrl Pts',(-19.6446081145374,21.1222351705132,
-5.65634279822551));
#108754=CARTESIAN_POINT('Ctrl Pts',(-19.6202911421272,21.1335629400343,
-5.65796373567001));
#108755=CARTESIAN_POINT('Ctrl Pts',(-19.6126184753653,21.1370814689355,
-5.65847217363576));
#108756=CARTESIAN_POINT('Ctrl Pts',(-19.5993943819441,21.1430503050897,
-5.65934338313637));
#108757=CARTESIAN_POINT('Ctrl Pts',(-19.5938531312243,21.1455227865318,
-5.65970691439905));
#108758=CARTESIAN_POINT('Ctrl Pts',(-19.5828196169244,21.1503891181994,
-5.66042776097299));
#108759=CARTESIAN_POINT('Ctrl Pts',(-19.577327670893,21.1527835447104,-5.66078509342141));
#108760=CARTESIAN_POINT('Ctrl Pts',(-19.5629365444683,21.1589853425098,
-5.6617176544521));
#108761=CARTESIAN_POINT('Ctrl Pts',(-19.5540212214647,21.1627550795279,
-5.66229159681302));
#108762=CARTESIAN_POINT('Ctrl Pts',(-19.523102918332,21.1755792635213,-5.66426925577876));
#108763=CARTESIAN_POINT('Ctrl Pts',(-19.5009728627888,21.1843240467543,
-5.66566250928614));
#108764=CARTESIAN_POINT('Ctrl Pts',(-19.3287272854687,21.2490520867295,
-5.67634629520721));
#108765=CARTESIAN_POINT('Ctrl Pts',(-19.1728412039705,21.2882053888621,
-5.68502830292001));
#108766=CARTESIAN_POINT('Ctrl Pts',(-18.8829078354626,21.3268947828466,
-5.70091667579017));
#108767=CARTESIAN_POINT('Ctrl Pts',(-18.750467595902,21.3320617312806,-5.70810129178447));
#108768=CARTESIAN_POINT('Ctrl Pts',(-18.6065505479636,21.3241936184566,
-5.71660684789848));
#108769=CARTESIAN_POINT('Ctrl Pts',(-18.5946733697303,21.3234437761401,
-5.7173140860814));
#108770=CARTESIAN_POINT('Ctrl Pts',(-18.5777949211286,21.3222352278593,
-5.71832745442766));
#108771=CARTESIAN_POINT('Ctrl Pts',(-18.5727877383108,21.3218587872043,
-5.71862912459734));
#108772=CARTESIAN_POINT('Ctrl Pts',(-18.5641599262325,21.3211792696706,
-5.71915079918951));
#108773=CARTESIAN_POINT('Ctrl Pts',(-18.5605386127916,21.3208846764226,
-5.71937032841991));
#108774=CARTESIAN_POINT('Ctrl Pts',(-18.5535178032749,21.3202953373065,
-5.71979707054641));
#108775=CARTESIAN_POINT('Ctrl Pts',(-18.5501182541012,21.3200016942763,
-5.72000421498617));
#108776=CARTESIAN_POINT('Ctrl Pts',(-18.5409461584418,21.3191870904055,
-5.72056445063816));
#108777=CARTESIAN_POINT('Ctrl Pts',(-18.5351750669417,21.3186506442176,
-5.72091839850437));
#108778=CARTESIAN_POINT('Ctrl Pts',(-18.5137519313256,21.3165705067397,
-5.72223749707443));
#108779=CARTESIAN_POINT('Ctrl Pts',(-18.4981154814572,21.3148761444119,
-5.72321058726142));
#108780=CARTESIAN_POINT('Ctrl Pts',(-18.3497769522213,21.2971278016013,
-5.73253072918418));
#108781=CARTESIAN_POINT('Ctrl Pts',(-18.2188682292552,21.2687146627467,
-5.7414116018875));
#108782=CARTESIAN_POINT('Ctrl Pts',(-17.9416054217305,21.1804049336318,
-5.76063027322858));
#108783=CARTESIAN_POINT('Ctrl Pts',(-17.7974501093668,21.1160818426246,
-5.77086528931925));
#108784=CARTESIAN_POINT('Ctrl Pts',(-17.6433919414537,21.0255841769066,
-5.78183904219307));
#108785=CARTESIAN_POINT('Ctrl Pts',(-17.6252098497493,21.0145315708405,
-5.78313580139118));
#108786=CARTESIAN_POINT('Ctrl Pts',(-17.5995859739166,20.998421226839,-5.78496623610069));
#108787=CARTESIAN_POINT('Ctrl Pts',(-17.5920054856057,20.9935875455977,
-5.7855081192895));
#108788=CARTESIAN_POINT('Ctrl Pts',(-17.5789785459452,20.9851637431653,
-5.78644005772953));
#108789=CARTESIAN_POINT('Ctrl Pts',(-17.5735175177193,20.9815964974231,
-5.78683095712439));
#108790=CARTESIAN_POINT('Ctrl Pts',(-17.5630910410947,20.9747167675602,
-5.78757774363431));
#108791=CARTESIAN_POINT('Ctrl Pts',(-17.5581229520907,20.9714084172547,
-5.78793378060146));
#108792=CARTESIAN_POINT('Ctrl Pts',(-17.5452367186009,20.962748325783,-5.78885783909681));
#108793=CARTESIAN_POINT('Ctrl Pts',(-17.5373406472939,20.9573638607746,
-5.78942462063207));
#108794=CARTESIAN_POINT('Ctrl Pts',(-17.5105200522233,20.9388071214526,
-5.7913519872035));
#108795=CARTESIAN_POINT('Ctrl Pts',(-17.4917739676509,20.9253789480587,
-5.79270282020472));
#108796=CARTESIAN_POINT('Ctrl Pts',(-17.3330266496184,20.8076939522846,
-5.80418499218966));
#108797=CARTESIAN_POINT('Ctrl Pts',(-17.2061981499819,20.6868001741757,
-5.81357468432394));
#108798=CARTESIAN_POINT('Ctrl Pts',(-17.0401292948202,20.4838607140944,
-5.82784065594843));
#108799=CARTESIAN_POINT('Ctrl Pts',(-16.9888884612902,20.4126470561164,
-5.83263736680235));
#108800=CARTESIAN_POINT('Ctrl Pts',(-16.9219814317527,20.3063176510739,
-5.83980884853194));
#108801=CARTESIAN_POINT('Ctrl Pts',(-16.9026205671445,20.2736292943877,
-5.84201516170409));
#108802=CARTESIAN_POINT('Ctrl Pts',(-16.8804643955397,20.2338158365741,
-5.84472599626804));
#108803=CARTESIAN_POINT('Ctrl Pts',(-16.8768136002998,20.2271718089862,
-5.84517915070592));
#108804=CARTESIAN_POINT('Ctrl Pts',(-16.8712033153791,20.2168305126279,
-5.84588589785408));
#108805=CARTESIAN_POINT('Ctrl Pts',(-16.8692189267295,20.2131467240102,
-5.84613793434782));
#108806=CARTESIAN_POINT('Ctrl Pts',(-16.86556475507,20.2063147416167,-5.84660592255908));
#108807=CARTESIAN_POINT('Ctrl Pts',(-16.8638919949633,20.2031682056456,
-5.84682168166879));
#108808=CARTESIAN_POINT('Ctrl Pts',(-16.8601353965849,20.1960586256707,
-5.84730968562893));
#108809=CARTESIAN_POINT('Ctrl Pts',(-16.8580561940066,20.1920932085399,
-5.84758221662765));
#108810=CARTESIAN_POINT('Ctrl Pts',(-16.8519769960045,20.1804090937888,
-5.84838617153706));
#108811=CARTESIAN_POINT('Ctrl Pts',(-16.848012005372,20.1726724270002,-5.84891971676906));
#108812=CARTESIAN_POINT('Ctrl Pts',(-16.820301828012,20.1177725804081,-5.85271310695916));
#108813=CARTESIAN_POINT('Ctrl Pts',(-16.7982828544642,20.0697638383392,
-5.85606807119919));
#108814=CARTESIAN_POINT('Ctrl Pts',(-16.7720816975599,20.0064945790881,
-5.86049228171665));
#108815=CARTESIAN_POINT('Ctrl Pts',(-16.766241426347,19.9919361235487,-5.86151052440592));
#108816=CARTESIAN_POINT('Ctrl Pts',(-16.7421267843932,19.9298353542444,
-5.86585135097812));
#108817=CARTESIAN_POINT('Ctrl Pts',(-16.7254099322273,19.8817077066625,
-5.869208583509));
#108818=CARTESIAN_POINT('Ctrl Pts',(-16.6782974638417,19.7284428611841,
-5.87980028943694));
#108819=CARTESIAN_POINT('Ctrl Pts',(-16.65430310197,19.6215171239257,-5.88703521426393));
#108820=CARTESIAN_POINT('Ctrl Pts',(-16.6308108371743,19.4586376726489,
-5.89761332839874));
#108821=CARTESIAN_POINT('Ctrl Pts',(-16.6250743300697,19.4037755503269,
-5.90110487989195));
#108822=CARTESIAN_POINT('Ctrl Pts',(-16.6192531183309,19.3145010745006,
-5.90666584479976));
#108823=CARTESIAN_POINT('Ctrl Pts',(-16.6178530393138,19.2802033479213,
-5.90877375553695));
#108824=CARTESIAN_POINT('Ctrl Pts',(-16.6171093085936,19.2350762159063,
-5.91151142237625));
#108825=CARTESIAN_POINT('Ctrl Pts',(-16.6170139622384,19.2242659808238,
-5.91216454408876));
#108826=CARTESIAN_POINT('Ctrl Pts',(-16.6169934229573,19.2065569047683,
-5.91323018605293));
#108827=CARTESIAN_POINT('Ctrl Pts',(-16.6170191407032,19.1996584189663,
-5.91364423653605));
#108828=CARTESIAN_POINT('Ctrl Pts',(-16.6171342072677,19.1863037889918,
-5.91444376773099));
#108829=CARTESIAN_POINT('Ctrl Pts',(-16.6172193730737,19.1798476939327,
-5.91482937496355));
#108830=CARTESIAN_POINT('Ctrl Pts',(-16.6174842503578,19.164939769398,-5.91571772463919));
#108831=CARTESIAN_POINT('Ctrl Pts',(-16.617685053987,19.1564883886591,-5.91621980135753));
#108832=CARTESIAN_POINT('Ctrl Pts',(-16.6183613633517,19.1337584663539,
-5.91756614071017));
#108833=CARTESIAN_POINT('Ctrl Pts',(-16.6189307931224,19.1194830047645,
-5.91840746380878));
#108834=CARTESIAN_POINT('Ctrl Pts',(-16.6254695501611,18.9887920505441,
-5.92607338714303));
#108835=CARTESIAN_POINT('Ctrl Pts',(-16.640900093674,18.8730428279378,-5.93258287206407));
#108836=CARTESIAN_POINT('Ctrl Pts',(-16.700362160854,18.600878542959,-5.94783519675533));
#108837=CARTESIAN_POINT('Ctrl Pts',(-16.7529850934015,18.4471286309441,
-5.95639703814145));
#108838=CARTESIAN_POINT('Ctrl Pts',(-16.836973585782,18.2707362443149,-5.9676036359387));
#108839=CARTESIAN_POINT('Ctrl Pts',(-16.8520471684738,18.2409183517398,
-5.96955082452033));
#108840=CARTESIAN_POINT('Ctrl Pts',(-16.8712656670052,18.2050362344626,
-5.9719740953264));
#108841=CARTESIAN_POINT('Ctrl Pts',(-16.8747456172116,18.1986189307154,
-5.97241066143764));
#108842=CARTESIAN_POINT('Ctrl Pts',(-16.8802427763706,18.1886056753827,
-5.97309704809824));
#108843=CARTESIAN_POINT('Ctrl Pts',(-16.8822374561672,18.1849973295554,
-5.97334545325473));
#108844=CARTESIAN_POINT('Ctrl Pts',(-16.8859789753791,18.1782754296004,
-5.97381022747824));
#108845=CARTESIAN_POINT('Ctrl Pts',(-16.8877231542394,18.1751604593793,
-5.97402642625152));
#108846=CARTESIAN_POINT('Ctrl Pts',(-16.8917139493268,18.1680753061379,
-5.97452004226621));
#108847=CARTESIAN_POINT('Ctrl Pts',(-16.8939655151901,18.1641079791198,
-5.97479777461323));
#108848=CARTESIAN_POINT('Ctrl Pts',(-16.8998557044989,18.1538069909157,
-5.97552230358343));
#108849=CARTESIAN_POINT('Ctrl Pts',(-16.9035142815429,18.1474848914291,
-5.97597034067082));
#108850=CARTESIAN_POINT('Ctrl Pts',(-16.9270757699051,18.1072518826028,
-5.97884251541472));
#108851=CARTESIAN_POINT('Ctrl Pts',(-16.9478861388533,18.0738843938315,
-5.98131976352892));
#108852=CARTESIAN_POINT('Ctrl Pts',(-16.9763283964887,18.0309884496147,
-5.98461188090347));
#108853=CARTESIAN_POINT('Ctrl Pts',(-16.9831319684865,18.0209168723103,
-5.98539283862582));
#108854=CARTESIAN_POINT('Ctrl Pts',(-16.9904473522303,18.0102861589587,
-5.9862252610686));
#108855=CARTESIAN_POINT('Ctrl Pts',(-16.990873264747,18.0096679274835,-5.98627370009617));
#108856=CARTESIAN_POINT('Ctrl Pts',(-17.004264453133,17.9902521205601,-5.98779586557816));
#108857=CARTESIAN_POINT('Ctrl Pts',(-17.0175323814377,17.9716657798494,
-5.98928004239451));
#108858=CARTESIAN_POINT('Ctrl Pts',(-17.0582314791836,17.9165600515037,
-5.99375480662154));
#108859=CARTESIAN_POINT('Ctrl Pts',(-17.0865461054743,17.8807104110526,
-5.99676606348786));
#108860=CARTESIAN_POINT('Ctrl Pts',(-17.1865154004732,17.7622286926707,
-6.00700644329614));
#108861=CARTESIAN_POINT('Ctrl Pts',(-17.263408736637,17.6842348938267,-6.01423702409776));
#108862=CARTESIAN_POINT('Ctrl Pts',(-17.3875659536343,17.5764246839066,
-6.02480601306636));
#108863=CARTESIAN_POINT('Ctrl Pts',(-17.4305385390984,17.5419553197506,
-6.02829281389283));
#108864=CARTESIAN_POINT('Ctrl Pts',(-17.5023719697226,17.4888045995001,
-6.03384709831494));
#108865=CARTESIAN_POINT('Ctrl Pts',(-17.5304270016017,17.4690824198566,
-6.03595296402337));
#108866=CARTESIAN_POINT('Ctrl Pts',(-17.5679391542238,17.4440512496766,
-6.03868840355027));
#108867=CARTESIAN_POINT('Ctrl Pts',(-17.5769741499679,17.4381218396458,
-6.03934129545955));
#108868=CARTESIAN_POINT('Ctrl Pts',(-17.5918497670957,17.4285215506393,
-6.04040665856749));
#108869=CARTESIAN_POINT('Ctrl Pts',(-17.5976635460145,17.4248096288317,
-6.04082065845261));
#108870=CARTESIAN_POINT('Ctrl Pts',(-17.6089545756466,17.417678086701,-6.04162015832602));
#108871=CARTESIAN_POINT('Ctrl Pts',(-17.6144295268518,17.4142549850751,
-6.04200578448717));
#108872=CARTESIAN_POINT('Ctrl Pts',(-17.6271101530793,17.4064071471837,
-6.04289427263789));
#108873=CARTESIAN_POINT('Ctrl Pts',(-17.6343268786544,17.4020004071293,
-6.04339646823619));
#108874=CARTESIAN_POINT('Ctrl Pts',(-17.6538130492785,17.3902612908354,
-6.0447433369212));
#108875=CARTESIAN_POINT('Ctrl Pts',(-17.6661308035135,17.3830096582104,
-6.0455850668113));
#108876=CARTESIAN_POINT('Ctrl Pts',(-17.7800282851797,17.3175008211735,
-6.05328245400493));
#108877=CARTESIAN_POINT('Ctrl Pts',(-17.8862102251636,17.2676372034031,
-6.05981988974111));
#108878=CARTESIAN_POINT('Ctrl Pts',(-18.1493512056869,17.1697625688518,
-6.0751882643298));
#108879=CARTESIAN_POINT('Ctrl Pts',(-18.3087951247446,17.1306988123705,
-6.08383351307016));
#108880=CARTESIAN_POINT('Ctrl Pts',(-18.5023525833226,17.1064765400254,
-6.09504687432979));
#108881=CARTESIAN_POINT('Ctrl Pts',(-18.5336629199799,17.1032655918991,
-6.09688399228954));
#108882=CARTESIAN_POINT('Ctrl Pts',(-18.5721758845913,17.1001818342797,
-6.09918480224686));
#108883=CARTESIAN_POINT('Ctrl Pts',(-18.5793232614034,17.0996460561393,
-6.09961352810246));
#108884=CARTESIAN_POINT('Ctrl Pts',(-18.5905569766248,17.0988613070054,
-6.10029028172232));
#108885=CARTESIAN_POINT('Ctrl Pts',(-18.5946416279887,17.0985878709642,
-6.10053695862382));
#108886=CARTESIAN_POINT('Ctrl Pts',(-18.6022940394019,17.0980978925119,
-6.10100027229927));
#108887=CARTESIAN_POINT('Ctrl Pts',(-18.605861563443,17.0978785372606,-6.10121674962493));
#108888=CARTESIAN_POINT('Ctrl Pts',(-18.6140274898488,17.0973971965551,
-6.10171335169056));
#108889=CARTESIAN_POINT('Ctrl Pts',(-18.618626188686,17.0971411833665,-6.10199380663432));
#108890=CARTESIAN_POINT('Ctrl Pts',(-18.632837179259,17.0963965574835,-6.10286283766763));
#108891=CARTESIAN_POINT('Ctrl Pts',(-18.6424518385142,17.0959584965065,
-6.10345413354853));
#108892=CARTESIAN_POINT('Ctrl Pts',(-18.738598852769,17.0922346736948,-6.10939825158321));
#108893=CARTESIAN_POINT('Ctrl Pts',(-18.8252434011508,17.0941960822023,
-6.11500406507168));
#108894=CARTESIAN_POINT('Ctrl Pts',(-19.0379880080281,17.1120980439608,
-6.12902170527436));
#108895=CARTESIAN_POINT('Ctrl Pts',(-19.1632593892837,17.1340941089328,
-6.13748308260308));
#108896=CARTESIAN_POINT('Ctrl Pts',(-19.379010787905,17.1923444584453,-6.1519473104327));
#108897=CARTESIAN_POINT('Ctrl Pts',(-19.4703935159452,17.223856764454,-6.15804199020151));
#108898=CARTESIAN_POINT('Ctrl Pts',(-19.572782778184,17.2672031314735,-6.16482092097132));
#108899=CARTESIAN_POINT('Ctrl Pts',(-19.5861890639793,17.2730431813018,
-6.16570768030029));
#108900=CARTESIAN_POINT('Ctrl Pts',(-19.6065883434729,17.2821821407976,
-6.16705594888665));
#108901=CARTESIAN_POINT('Ctrl Pts',(-19.6136253618458,17.2853811445636,
-6.16752086249995));
#108902=CARTESIAN_POINT('Ctrl Pts',(-19.6264196544637,17.2912821551568,
-6.16836584596404));
#108903=CARTESIAN_POINT('Ctrl Pts',(-19.6321825512969,17.2939716878995,
-6.16874633967788));
#108904=CARTESIAN_POINT('Ctrl Pts',(-19.644624184719,17.299846593227,-6.16956759669094));
#108905=CARTESIAN_POINT('Ctrl Pts',(-19.6512985329181,17.303041102735,-6.17000803772745));
#108906=CARTESIAN_POINT('Ctrl Pts',(-19.6694152812477,17.31182926927,-6.17120331116676));
#108907=CARTESIAN_POINT('Ctrl Pts',(-19.6808242875425,17.3174913541168,
-6.17195575586583));
#108908=CARTESIAN_POINT('Ctrl Pts',(-19.7368646384045,17.345936335266,-6.17565125888036));
#108909=CARTESIAN_POINT('Ctrl Pts',(-19.7807305081523,17.3701969738104,
-6.17854195084981));
#108910=CARTESIAN_POINT('Ctrl Pts',(-19.9725202030574,17.4853439778855,
-6.19124131817274));
#108911=CARTESIAN_POINT('Ctrl Pts',(-20.1097822100573,17.5926538725432,
-6.20043480306611));
#108912=CARTESIAN_POINT('Ctrl Pts',(-20.2767028355463,17.7599007239427,
-6.21342104815364));
#108913=CARTESIAN_POINT('Ctrl Pts',(-20.3190029643256,17.80622756216,-6.21691353812115));
#108914=CARTESIAN_POINT('Ctrl Pts',(-20.3790002901429,17.8781010943263,
-6.22229879364762));
#108915=CARTESIAN_POINT('Ctrl Pts',(-20.3982951629098,17.9022728202578,
-6.2241048180542));
#108916=CARTESIAN_POINT('Ctrl Pts',(-20.421376501477,17.9325242058161,-6.22637099027759));
#108917=CARTESIAN_POINT('Ctrl Pts',(-20.4256717674372,17.9382131199545,
-6.22679740542314));
#108918=CARTESIAN_POINT('Ctrl Pts',(-20.4323832437174,17.9471961994309,
-6.22747131891753));
#108919=CARTESIAN_POINT('Ctrl Pts',(-20.4348188353693,17.9504759115839,
-6.22771748517498));
#108920=CARTESIAN_POINT('Ctrl Pts',(-20.4393684431548,17.9566395019801,
-6.22818037679325));
#108921=CARTESIAN_POINT('Ctrl Pts',(-20.4414846510105,17.9595216934423,
-6.22839694594243));
#108922=CARTESIAN_POINT('Ctrl Pts',(-20.4463180504041,17.9661396730962,
-6.2288944736895));
#108923=CARTESIAN_POINT('Ctrl Pts',(-20.4490303152467,17.9698789921648,
-6.2291757671354));
#108924=CARTESIAN_POINT('Ctrl Pts',(-20.4573967030695,17.9814932743113,
-6.23004993459246));
#108925=CARTESIAN_POINT('Ctrl Pts',(-20.4630088932696,17.9893980912523,
-6.23064557410465));
#108926=CARTESIAN_POINT('Ctrl Pts',(-20.525858317636,18.0792227489039,-6.23741895062477));
#108927=CARTESIAN_POINT('Ctrl Pts',(-20.5772738131753,18.1650492918994,
-6.24393187552144));
#108928=CARTESIAN_POINT('Ctrl Pts',(-20.6603886046325,18.3290879047529,
-6.25604814573764));
#108929=CARTESIAN_POINT('Ctrl Pts',(-20.6938230869984,18.4061322178279,
-6.26161630673243));
#108930=CARTESIAN_POINT('Ctrl Pts',(-20.7225804911066,18.4848893814367,
-6.26710637686285));
#108931=CARTESIAN_POINT('',(-20.8509997150786,19.2120983429817,-5.28730630211274));
#108932=CARTESIAN_POINT('Ctrl Pts',(-20.7225806138063,18.4848897174713,
-6.04247212253779));
#108933=CARTESIAN_POINT('Ctrl Pts',(-20.7198614621432,18.477442842784,-6.04199082365182));
#108934=CARTESIAN_POINT('Ctrl Pts',(-20.7171004599269,18.4700111880572,
-6.04151092132984));
#108935=CARTESIAN_POINT('Ctrl Pts',(-20.7114649079107,18.4550993790409,
-6.04054876329006));
#108936=CARTESIAN_POINT('Ctrl Pts',(-20.7085895172297,18.4476197199386,
-6.04006654790803));
#108937=CARTESIAN_POINT('Ctrl Pts',(-20.7033486788313,18.434214648031,-6.03920297565442));
#108938=CARTESIAN_POINT('Ctrl Pts',(-20.7009987945502,18.4282832916904,
-6.03882110180472));
#108939=CARTESIAN_POINT('Ctrl Pts',(-20.6959425293938,18.4156873251404,
-6.03801060091683));
#108940=CARTESIAN_POINT('Ctrl Pts',(-20.6932289167103,18.40902569036,-6.03758222352211));
#108941=CARTESIAN_POINT('Ctrl Pts',(-20.6858435948529,18.3911567184248,
-6.03643381295184));
#108942=CARTESIAN_POINT('Ctrl Pts',(-20.6811092890116,18.3799754209312,
-6.03571590704927));
#108943=CARTESIAN_POINT('Ctrl Pts',(-20.657153366327,18.324726032539,-6.03217125619475));
#108944=CARTESIAN_POINT('Ctrl Pts',(-20.6365297918646,18.2812788987519,
-6.02939279002619));
#108945=CARTESIAN_POINT('Ctrl Pts',(-20.537431340742,18.0896467430304,-6.01711812413672));
#108946=CARTESIAN_POINT('Ctrl Pts',(-20.4430052929719,17.9504048372787,
-6.00819989208419));
#108947=CARTESIAN_POINT('Ctrl Pts',(-20.2684509412495,17.74918797159,-5.99361602285774));
#108948=CARTESIAN_POINT('Ctrl Pts',(-20.1986342586465,17.6792443202059,
-5.98812327491185));
#108949=CARTESIAN_POINT('Ctrl Pts',(-20.1168931575858,17.6080684639141,
-5.98170202225121));
#108950=CARTESIAN_POINT('Ctrl Pts',(-20.1095379825726,17.6017522735439,
-5.98112428390987));
#108951=CARTESIAN_POINT('Ctrl Pts',(-20.0986146031857,17.5925015214897,
-5.98026590102706));
#108952=CARTESIAN_POINT('Ctrl Pts',(-20.0950796404054,17.5895276592817,
-5.97998805981999));
#108953=CARTESIAN_POINT('Ctrl Pts',(-20.0887912538401,17.5842724738487,
-5.97949364733824));
#108954=CARTESIAN_POINT('Ctrl Pts',(-20.0860417540153,17.5819865313602,
-5.97927741804499));
#108955=CARTESIAN_POINT('Ctrl Pts',(-20.0801385590092,17.577103837967,-5.97881303717233));
#108956=CARTESIAN_POINT('Ctrl Pts',(-20.0769831827091,17.5745092854936,
-5.97856473934054));
#108957=CARTESIAN_POINT('Ctrl Pts',(-20.0683014444765,17.5674126231789,
-5.97788140683934));
#108958=CARTESIAN_POINT('Ctrl Pts',(-20.0627598819095,17.5629293149645,
-5.97744505464086));
#108959=CARTESIAN_POINT('Ctrl Pts',(-20.0330577929898,17.53914652113,-5.9751057905538));
#108960=CARTESIAN_POINT('Ctrl Pts',(-20.0085005702278,17.5203512287885,
-5.97317010611272));
#108961=CARTESIAN_POINT('Ctrl Pts',(-19.932933748562,17.4650969610725,-5.9672307357491));
#108962=CARTESIAN_POINT('Ctrl Pts',(-19.8807099036406,17.4303611109995,
-5.96314961963098));
#108963=CARTESIAN_POINT('Ctrl Pts',(-19.7118261345998,17.3285442591615,
-5.95019059956498));
#108964=CARTESIAN_POINT('Ctrl Pts',(-19.5902575770625,17.2702239376253,
-5.94122494624613));
#108965=CARTESIAN_POINT('Ctrl Pts',(-19.4256423302445,17.2097535373328,
-5.92993149527873));
#108966=CARTESIAN_POINT('Ctrl Pts',(-19.3869104091957,17.1967843128682,
-5.92732954855638));
#108967=CARTESIAN_POINT('Ctrl Pts',(-19.3014161498651,17.1708824909948,
-5.92171057413525));
#108968=CARTESIAN_POINT('Ctrl Pts',(-19.2545345789874,17.1584199420785,
-5.91870896433799));
#108969=CARTESIAN_POINT('Ctrl Pts',(-19.1949880124128,17.1447624393269,
-5.91499309747588));
#108970=CARTESIAN_POINT('Ctrl Pts',(-19.1826878248616,17.1420565857681,
-5.91423062934022));
#108971=CARTESIAN_POINT('Ctrl Pts',(-19.1631556905309,17.1379421959932,
-5.91302775897249));
#108972=CARTESIAN_POINT('Ctrl Pts',(-19.1559394234829,17.1364614029822,
-5.91258505135177));
#108973=CARTESIAN_POINT('Ctrl Pts',(-19.1424772954541,17.1337720954769,
-5.91176228633943));
#108974=CARTESIAN_POINT('Ctrl Pts',(-19.1362334512421,17.1325540131389,
-5.91138192725712));
#108975=CARTESIAN_POINT('Ctrl Pts',(-19.1223512231174,17.1299106935208,
-5.91053898161985));
#108976=CARTESIAN_POINT('Ctrl Pts',(-19.1147102678429,17.1284993232986,
-5.91007684170201));
#108977=CARTESIAN_POINT('Ctrl Pts',(-19.092479206305,17.1245194414676,-5.90873746286848));
#108978=CARTESIAN_POINT('Ctrl Pts',(-19.0778695078084,17.1220619346721,
-5.90786375536702));
#108979=CARTESIAN_POINT('Ctrl Pts',(-18.961238213152,17.1037000734621,-5.90093813149453));
#108980=CARTESIAN_POINT('Ctrl Pts',(-18.8581967084162,17.0951244404664,
-5.89512924265497));
#108981=CARTESIAN_POINT('Ctrl Pts',(-18.595291539024,17.0925251571705,-5.88065391693254));
#108982=CARTESIAN_POINT('Ctrl Pts',(-18.4360031144689,17.1090091203861,
-5.87222556514472));
#108983=CARTESIAN_POINT('Ctrl Pts',(-18.2326858998322,17.1536402720964,
-5.86047047933077));
#108984=CARTESIAN_POINT('Ctrl Pts',(-18.1856531319034,17.1656736688338,
-5.85767570280846));
#108985=CARTESIAN_POINT('Ctrl Pts',(-18.1316337524453,17.181491661299,-5.85433398107354));
#108986=CARTESIAN_POINT('Ctrl Pts',(-18.1242001559643,17.1837128128721,
-5.85387119253759));
#108987=CARTESIAN_POINT('Ctrl Pts',(-18.1123333379977,17.1873297793388,
-5.85312745923925));
#108988=CARTESIAN_POINT('Ctrl Pts',(-18.1078921331725,17.188699444002,-5.85284800153556));
#108989=CARTESIAN_POINT('Ctrl Pts',(-18.1000300526545,17.1911524854589,
-5.85235125666072));
#108990=CARTESIAN_POINT('Ctrl Pts',(-18.0966073787929,17.1922299481115,
-5.85213431800261));
#108991=CARTESIAN_POINT('Ctrl Pts',(-18.0893538418128,17.1945336577665,
-5.85167309128154));
#108992=CARTESIAN_POINT('Ctrl Pts',(-18.0855237891369,17.1957621028903,
-5.85142868092559));
#108993=CARTESIAN_POINT('Ctrl Pts',(-18.0751860252404,17.1991103432874,
-5.85076667849918));
#108994=CARTESIAN_POINT('Ctrl Pts',(-18.0686851205157,17.2012507737768,
-5.85034790003425));
#108995=CARTESIAN_POINT('Ctrl Pts',(-18.0363453407776,17.2120727886043,
-5.84825265757752));
#108996=CARTESIAN_POINT('Ctrl Pts',(-18.0106667357245,17.2212209053297,
-5.84655085670326));
#108997=CARTESIAN_POINT('Ctrl Pts',(-17.9367518163412,17.2491732257531,
-5.84155546591997));
#108998=CARTESIAN_POINT('Ctrl Pts',(-17.889021345343,17.2692535411416,-5.83820866876273));
#108999=CARTESIAN_POINT('Ctrl Pts',(-17.7166743288491,17.3493186293195,
-5.82578656298283));
#109000=CARTESIAN_POINT('Ctrl Pts',(-17.5972690262176,17.4197278828816,
-5.81654003223718));
#109001=CARTESIAN_POINT('Ctrl Pts',(-17.4079534444384,17.557963641679,-5.80136173524123));
#109002=CARTESIAN_POINT('Ctrl Pts',(-17.3342656355115,17.6198756040067,
-5.79528901843943));
#109003=CARTESIAN_POINT('Ctrl Pts',(-17.2550407733338,17.6962191095029,
-5.78857468787628));
#109004=CARTESIAN_POINT('Ctrl Pts',(-17.2451437466784,17.7059456449375,
-5.78773215837909));
#109005=CARTESIAN_POINT('Ctrl Pts',(-17.2294565675115,17.7216687688662,
-5.78639044133519));
#109006=CARTESIAN_POINT('Ctrl Pts',(-17.2236050824061,17.7276033395333,
-5.78588853788793));
#109007=CARTESIAN_POINT('Ctrl Pts',(-17.213296031286,17.7381830114306,-5.78500168230809));
#109008=CARTESIAN_POINT('Ctrl Pts',(-17.2088243498558,17.7428141534846,
-5.78461611337973));
#109009=CARTESIAN_POINT('Ctrl Pts',(-17.199569512493,17.7524869306145,-5.78381623301755));
#109010=CARTESIAN_POINT('Ctrl Pts',(-17.194789911567,17.757531871696,-5.7834020782515));
#109011=CARTESIAN_POINT('Ctrl Pts',(-17.1824805137973,17.7706534409504,
-5.7823326330014));
#109012=CARTESIAN_POINT('Ctrl Pts',(-17.1749888490189,17.7787656740823,
-5.78167898108254));
#109013=CARTESIAN_POINT('Ctrl Pts',(-17.143079395792,17.813865378173,-5.7788823463047));
#109014=CARTESIAN_POINT('Ctrl Pts',(-17.1192954062883,17.8414223903696,
-5.77676607225918));
#109015=CARTESIAN_POINT('Ctrl Pts',(-17.0583345653391,17.9158507505079,
-5.77124096245622));
#109016=CARTESIAN_POINT('Ctrl Pts',(-17.0224126007662,17.96370869685,-5.76787962242608));
#109017=CARTESIAN_POINT('Ctrl Pts',(-16.8936198752804,18.1513585474914,
-5.75527051065746));
#109018=CARTESIAN_POINT('Ctrl Pts',(-16.8154661405173,18.3004731198014,
-5.74643984015733));
#109019=CARTESIAN_POINT('Ctrl Pts',(-16.7365386377461,18.5076195074023,
-5.73397914262836));
#109020=CARTESIAN_POINT('Ctrl Pts',(-16.7192749236401,18.5587133844757,
-5.73088659255996));
#109021=CARTESIAN_POINT('Ctrl Pts',(-16.7015015511334,18.6187876510889,
-5.72716901417719));
#109022=CARTESIAN_POINT('Ctrl Pts',(-16.6990736176738,18.6271849407554,
-5.72664753855623));
#109023=CARTESIAN_POINT('Ctrl Pts',(-16.6954780245903,18.6399156840981,
-5.72585385932323));
#109024=CARTESIAN_POINT('Ctrl Pts',(-16.6942719918172,18.6442383288546,
-5.72558383249738));
#109025=CARTESIAN_POINT('Ctrl Pts',(-16.6921327836786,18.6520009168243,
-5.72509790112799));
#109026=CARTESIAN_POINT('Ctrl Pts',(-16.6911945435307,18.6554394085201,
-5.72488229420803));
#109027=CARTESIAN_POINT('Ctrl Pts',(-16.6891757635245,18.6629121564715,
-5.72441292972801));
#109028=CARTESIAN_POINT('Ctrl Pts',(-16.6880984910884,18.6669471924167,
-5.72415899218083));
#109029=CARTESIAN_POINT('Ctrl Pts',(-16.6851086425479,18.6782804419156,
-5.72344441532025));
#109030=CARTESIAN_POINT('Ctrl Pts',(-16.6832231535289,18.6855856451814,
-5.72298225567902));
#109031=CARTESIAN_POINT('Ctrl Pts',(-16.6722351572208,18.7291182533743,
-5.72021958464714));
#109032=CARTESIAN_POINT('Ctrl Pts',(-16.6640543255889,18.7655689798445,
-5.71787102464256));
#109033=CARTESIAN_POINT('Ctrl Pts',(-16.6403977670609,18.8857747405225,
-5.71005239539296));
#109034=CARTESIAN_POINT('Ctrl Pts',(-16.6290112838938,18.9702461485174,
-5.70444490279422));
#109035=CARTESIAN_POINT('Ctrl Pts',(-16.6096334004436,19.2327823223064,
-5.68705420474811));
#109036=CARTESIAN_POINT('Ctrl Pts',(-16.6189869202772,19.4113798457865,
-5.67535026087291));
#109037=CARTESIAN_POINT('Ctrl Pts',(-16.6546513085106,19.6091421928189,
-5.66298375792962));
#109038=CARTESIAN_POINT('Ctrl Pts',(-16.6590571167547,19.6315000374013,
-5.66159295495752));
#109039=CARTESIAN_POINT('Ctrl Pts',(-16.6658127329985,19.6630850734839,
-5.6596378324023));
#109040=CARTESIAN_POINT('Ctrl Pts',(-16.6678649975143,19.6723736459497,
-5.6590640565413));
#109041=CARTESIAN_POINT('Ctrl Pts',(-16.6713049976595,19.6874597120256,
-5.65813401181504));
#109042=CARTESIAN_POINT('Ctrl Pts',(-16.6726547189639,19.6932656564005,
-5.65777652800008));
#109043=CARTESIAN_POINT('Ctrl Pts',(-16.6755343998046,19.7054198747651,
-5.65702907849844));
#109044=CARTESIAN_POINT('Ctrl Pts',(-16.6770692481107,19.711766934967,-5.6566392744995));
#109045=CARTESIAN_POINT('Ctrl Pts',(-16.6807963422214,19.7268733067208,
-5.65571271409452));
#109046=CARTESIAN_POINT('Ctrl Pts',(-16.6830153204296,19.7356259399958,
-5.65517682577423));
#109047=CARTESIAN_POINT('Ctrl Pts',(-16.6907089317176,19.7651779347203,
-5.65337052474706));
#109048=CARTESIAN_POINT('Ctrl Pts',(-16.6964446151451,19.7859084073686,
-5.65210855789065));
#109049=CARTESIAN_POINT('Ctrl Pts',(-16.7531069261878,19.9791920036931,
-5.64038142589846));
#109050=CARTESIAN_POINT('Ctrl Pts',(-16.825516469301,20.1446776122042,-5.63071760710449));
#109051=CARTESIAN_POINT('Ctrl Pts',(-16.9796612851757,20.4019591023959,
-5.61439336705209));
#109052=CARTESIAN_POINT('Ctrl Pts',(-17.0499641430449,20.4994497497098,
-5.60780805151875));
#109053=CARTESIAN_POINT('Ctrl Pts',(-17.1343293722125,20.597662673797,-5.60013489953289));
#109054=CARTESIAN_POINT('Ctrl Pts',(-17.1405762171617,20.6048364785569,
-5.59956790063481));
#109055=CARTESIAN_POINT('Ctrl Pts',(-17.1499045671602,20.6154043833545,
-5.59872249052285));
#109056=CARTESIAN_POINT('Ctrl Pts',(-17.1529491910044,20.6188310803491,
-5.59844676183229));
#109057=CARTESIAN_POINT('Ctrl Pts',(-17.158386179031,20.6249104807088,-5.5979546715447));
#109058=CARTESIAN_POINT('Ctrl Pts',(-17.1607741516917,20.6275670440444,
-5.59773863996061));
#109059=CARTESIAN_POINT('Ctrl Pts',(-17.1659229072422,20.6332658358075,
-5.59727304572888));
#109060=CARTESIAN_POINT('Ctrl Pts',(-17.1686857844283,20.6363060311397,
-5.59702332823503));
#109061=CARTESIAN_POINT('Ctrl Pts',(-17.1763371418638,20.6446762980538,
-5.59633216816887));
#109062=CARTESIAN_POINT('Ctrl Pts',(-17.1812440605447,20.6499893315196,
-5.59588935846801));
#109063=CARTESIAN_POINT('Ctrl Pts',(-17.2082840034164,20.6789678563894,
-5.59345214687355));
#109064=CARTESIAN_POINT('Ctrl Pts',(-17.2309296210877,20.7021465721444,
-5.59142170700483));
#109065=CARTESIAN_POINT('Ctrl Pts',(-17.3705213873353,20.8386130813369,
-5.57901857875062));
#109066=CARTESIAN_POINT('Ctrl Pts',(-17.4996839447417,20.9386174512351,
-5.56805381332734));
#109067=CARTESIAN_POINT('Ctrl Pts',(-17.7390295010385,21.0832646383837,
-5.54978643656016));
#109068=CARTESIAN_POINT('Ctrl Pts',(-17.8438727455666,21.1353238949974,
-5.54234351682457));
#109069=CARTESIAN_POINT('Ctrl Pts',(-17.9657760155113,21.183745593241,-5.53433437114166));
#109070=CARTESIAN_POINT('Ctrl Pts',(-17.9791120156076,21.1888871081894,
-5.53346622149141));
#109071=CARTESIAN_POINT('Ctrl Pts',(-18.0004190293026,21.1968548416351,
-5.53209169083875));
#109072=CARTESIAN_POINT('Ctrl Pts',(-18.0083564952692,21.1997689659428,
-5.53158238029628));
#109073=CARTESIAN_POINT('Ctrl Pts',(-18.0223857892135,21.2048244421099,
-5.53068694405578));
#109074=CARTESIAN_POINT('Ctrl Pts',(-18.028470314185,21.2069856098717,-5.53030016196275));
#109075=CARTESIAN_POINT('Ctrl Pts',(-18.0410750656224,21.2113978639122,
-5.52950210424154));
#109076=CARTESIAN_POINT('Ctrl Pts',(-18.0475966044011,21.2136449907232,
-5.5290909638539));
#109077=CARTESIAN_POINT('Ctrl Pts',(-18.0643637429713,21.2193309183333,
-5.52803836246365));
#109078=CARTESIAN_POINT('Ctrl Pts',(-18.0746249828955,21.2227232383295,
-5.52739844213928));
#109079=CARTESIAN_POINT('Ctrl Pts',(-18.1175522224221,21.236551054962,-5.52473863686662));
#109080=CARTESIAN_POINT('Ctrl Pts',(-18.1504444476018,21.2462710021974,
-5.5227422612433));
#109081=CARTESIAN_POINT('Ctrl Pts',(-18.2367413468168,21.2695082426363,
-5.51760055973521));
#109082=CARTESIAN_POINT('Ctrl Pts',(-18.2904639391543,21.2817483575811,
-5.51449457513981));
#109083=CARTESIAN_POINT('Ctrl Pts',(-18.4520628622403,21.3119882915455,
-5.50535291137145));
#109084=CARTESIAN_POINT('Ctrl Pts',(-18.5609189914801,21.3237432881816,
-5.49946597068928));
#109085=CARTESIAN_POINT('Ctrl Pts',(-18.7134445135988,21.3283423530161,
-5.49115818590459));
#109086=CARTESIAN_POINT('Ctrl Pts',(-18.7567221411009,21.3283201641636,
-5.48879290318467));
#109087=CARTESIAN_POINT('Ctrl Pts',(-18.8752016225692,21.3246264537201,
-5.48222974381557));
#109088=CARTESIAN_POINT('Ctrl Pts',(-18.9502490327657,21.3182703889049,
-5.4779757947743));
#109089=CARTESIAN_POINT('Ctrl Pts',(-19.034186345117,21.3066304913513,-5.472953445476));
#109090=CARTESIAN_POINT('Ctrl Pts',(-19.0435740917873,21.305264279453,-5.47238796482603));
#109091=CARTESIAN_POINT('Ctrl Pts',(-19.0574787294372,21.3031451855739,
-5.47154439022515));
#109092=CARTESIAN_POINT('Ctrl Pts',(-19.0620030198026,21.302440647978,-5.4712689619221));
#109093=CARTESIAN_POINT('Ctrl Pts',(-19.0700522777361,21.3011604300814,
-5.47077720018088));
#109094=CARTESIAN_POINT('Ctrl Pts',(-19.0735781089767,21.3005905016347,
-5.47056119505293));
#109095=CARTESIAN_POINT('Ctrl Pts',(-19.0811596414179,21.2993452989248,
-5.4700954207417));
#109096=CARTESIAN_POINT('Ctrl Pts',(-19.0852147633053,21.2986671414626,
-5.46984549546054));
#109097=CARTESIAN_POINT('Ctrl Pts',(-19.0964127235129,21.2967609034773,
-5.46915318776421));
#109098=CARTESIAN_POINT('Ctrl Pts',(-19.1035511916393,21.2955079615817,
-5.46870943088116));
#109099=CARTESIAN_POINT('Ctrl Pts',(-19.1427887234668,21.2884131174835,
-5.46625743888596));
#109100=CARTESIAN_POINT('Ctrl Pts',(-19.1747539975205,21.281866756592,-5.46421265903628));
#109101=CARTESIAN_POINT('Ctrl Pts',(-19.3650776320553,21.2382833653326,
-5.45180470637538));
#109102=CARTESIAN_POINT('Ctrl Pts',(-19.5188868831278,21.1838378908713,
-5.44085307670154));
#109103=CARTESIAN_POINT('Ctrl Pts',(-19.7698225600987,21.0609720412171,
-5.4226029810598));
#109104=CARTESIAN_POINT('Ctrl Pts',(-19.8702833837605,21.0010259214969,
-5.41516465564124));
#109105=CARTESIAN_POINT('Ctrl Pts',(-19.9769292840044,20.924773661339,-5.40715950387927));
#109106=CARTESIAN_POINT('Ctrl Pts',(-19.9884739256701,20.9163411837187,
-5.40629113600111));
#109107=CARTESIAN_POINT('Ctrl Pts',(-20.0067103295512,20.9027354778578,
-5.40491632623092));
#109108=CARTESIAN_POINT('Ctrl Pts',(-20.0134578828898,20.8976380877775,
-5.40440695294765));
#109109=CARTESIAN_POINT('Ctrl Pts',(-20.0253035015431,20.8885774080583,
-5.40351144372293));
#109110=CARTESIAN_POINT('Ctrl Pts',(-20.030414282376,20.884630993681,-5.4031246510499));
#109111=CARTESIAN_POINT('Ctrl Pts',(-20.0407754087462,20.8765544581456,
-5.4023395953425));
#109112=CARTESIAN_POINT('Ctrl Pts',(-20.0460244242168,20.8724227438505,
-5.40194140165657));
#109113=CARTESIAN_POINT('Ctrl Pts',(-20.0593328865063,20.8618447070201,
-5.40093053084449));
#109114=CARTESIAN_POINT('Ctrl Pts',(-20.0673649720068,20.8553641214436,
-5.40031923123136));
#109115=CARTESIAN_POINT('Ctrl Pts',(-20.0846849211483,20.8411793918405,
-5.39899822040494));
#109116=CARTESIAN_POINT('Ctrl Pts',(-20.093954985742,20.83345402137,-5.39828938423295));
#109117=CARTESIAN_POINT('Ctrl Pts',(-20.1204060637922,20.8110245606152,
-5.39626109780758));
#109118=CARTESIAN_POINT('Ctrl Pts',(-20.1374184930236,20.796123640981,-5.39494957154413));
#109119=CARTESIAN_POINT('Ctrl Pts',(-20.1946136016826,20.7443845712997,
-5.39051143173487));
#109120=CARTESIAN_POINT('Ctrl Pts',(-20.2336122123264,20.7062672595046,
-5.38743606980876));
#109121=CARTESIAN_POINT('Ctrl Pts',(-20.3459462182262,20.587650653921,-5.37834788157023));
#109122=CARTESIAN_POINT('Ctrl Pts',(-20.4145892434939,20.5029591200392,
-5.37248395855781));
#109123=CARTESIAN_POINT('Ctrl Pts',(-20.5445159918407,20.3146748968004,
-5.36003273210043));
#109124=CARTESIAN_POINT('Ctrl Pts',(-20.6041001691299,20.2103915264019,
-5.35345196348697));
#109125=CARTESIAN_POINT('Ctrl Pts',(-20.6585345816035,20.0930125806035,
-5.34578397365668));
#109126=CARTESIAN_POINT('Ctrl Pts',(-20.6624795982953,20.0843532958917,
-5.34521678977393));
#109127=CARTESIAN_POINT('Ctrl Pts',(-20.6682385290129,20.0714831961549,
-5.34437115604783));
#109128=CARTESIAN_POINT('Ctrl Pts',(-20.6700974197501,20.067292472414,-5.34409539078719));
#109129=CARTESIAN_POINT('Ctrl Pts',(-20.6733804847907,20.0598257158696,
-5.34360326047251));
#109130=CARTESIAN_POINT('Ctrl Pts',(-20.6748099943035,20.0565520838434,
-5.34338722563867));
#109131=CARTESIAN_POINT('Ctrl Pts',(-20.6778655301907,20.0495062156744,
-5.34292165319898));
#109132=CARTESIAN_POINT('Ctrl Pts',(-20.679488841256,20.0457329160121,-5.3426719608987));
#109133=CARTESIAN_POINT('Ctrl Pts',(-20.6839392340168,20.0353047155353,
-5.34198093994415));
#109134=CARTESIAN_POINT('Ctrl Pts',(-20.6867431878243,20.0286400915702,
-5.34153824504982));
#109135=CARTESIAN_POINT('Ctrl Pts',(-20.7019150576371,19.9920553797923,
-5.33910281758421));
#109136=CARTESIAN_POINT('Ctrl Pts',(-20.7136287844909,19.9618706883165,
-5.33707410796012));
#109137=CARTESIAN_POINT('Ctrl Pts',(-20.7800606006944,19.7783109685087,
-5.32467155729117));
#109138=CARTESIAN_POINT('Ctrl Pts',(-20.8176233577576,19.6193127826616,
-5.31370520091951));
#109139=CARTESIAN_POINT('Ctrl Pts',(-20.8461452897875,19.3761078302404,
-5.29771008832249));
#109140=CARTESIAN_POINT('Ctrl Pts',(-20.8509571489542,19.2941423626708,
-5.29243882933731));
#109141=CARTESIAN_POINT('Ctrl Pts',(-20.8509997150786,19.2120983429817,
-5.28730630211274));
#109142=CARTESIAN_POINT('Ctrl Pts',(-20.8509997162508,19.212096081275,-5.28730616062444));
#109143=CARTESIAN_POINT('Ctrl Pts',(-20.8510131380423,19.1861728860207,
-5.28568445267461));
#109144=CARTESIAN_POINT('Ctrl Pts',(-20.8505504063707,19.1602505638564,
-5.28407676135363));
#109145=CARTESIAN_POINT('Ctrl Pts',(-20.848973668512,19.1167355904135,-5.2814009878188));
#109146=CARTESIAN_POINT('Ctrl Pts',(-20.8481159291783,19.0991372946227,
-5.28032517195835));
#109147=CARTESIAN_POINT('Ctrl Pts',(-20.8465415722552,19.0734384836758,
-5.27876307643348));
#109148=CARTESIAN_POINT('Ctrl Pts',(-20.8459978401128,19.065328480728,-5.27827141041774));
#109149=CARTESIAN_POINT('Ctrl Pts',(-20.8449526650894,19.0509780126566,
-5.27740366600639));
#109150=CARTESIAN_POINT('Ctrl Pts',(-20.8444702258813,19.0447363008249,
-5.27702699539688));
#109151=CARTESIAN_POINT('Ctrl Pts',(-20.8434611334825,19.0323936642418,
-5.27628361072404));
#109152=CARTESIAN_POINT('Ctrl Pts',(-20.8429356825822,19.0262927050715,
-5.27591686263781));
#109153=CARTESIAN_POINT('Ctrl Pts',(-20.8418361331652,19.0141428099679,
-5.27518787020845));
#109154=CARTESIAN_POINT('Ctrl Pts',(-20.8412624496712,19.008093896263,-5.27482561649629));
#109155=CARTESIAN_POINT('Ctrl Pts',(-20.8398285584689,18.9936373811815,
-5.273961440145));
#109156=CARTESIAN_POINT('Ctrl Pts',(-20.8389440263602,18.9852322548256,
-5.27346028624028));
#109157=CARTESIAN_POINT('Ctrl Pts',(-20.8360988523223,18.9596681874912,
-5.27193979154803));
#109158=CARTESIAN_POINT('Ctrl Pts',(-20.833978522619,18.9425274771431,-5.27092546456861));
#109159=CARTESIAN_POINT('Ctrl Pts',(-20.8260338111836,18.8841729794934,
-5.26748815691785));
#109160=CARTESIAN_POINT('Ctrl Pts',(-20.8192037342712,18.8431045235691,
-5.26509642151262));
#109161=CARTESIAN_POINT('Ctrl Pts',(-20.7899099159963,18.6942361451609,
-5.2564925000987));
#109162=CARTESIAN_POINT('Ctrl Pts',(-20.7602778853229,18.5881303508605,
-5.25049686993618));
#109163=CARTESIAN_POINT('Ctrl Pts',(-20.7225806829213,18.4848899067551,
-5.2445270986103));
#109164=CARTESIAN_POINT('Origin',(-18.734,19.211,0.));
#109165=CARTESIAN_POINT('',(-20.722580615654,18.4848897225317,-4.44630506752222));
#109166=CARTESIAN_POINT('',(-20.7225805995351,18.4848896783871,-4.66702134980151));
#109167=CARTESIAN_POINT('',(-20.7225806137986,18.4848897174502,0.));
#109168=CARTESIAN_POINT('Ctrl Pts',(-20.7225805995351,18.4848896783871,
-4.66702134980151));
#109169=CARTESIAN_POINT('Ctrl Pts',(-20.7691765746879,18.6125009372375,
-4.67446198781971));
#109170=CARTESIAN_POINT('Ctrl Pts',(-20.8033897591205,18.7443251558462,
-4.68169550656151));
#109171=CARTESIAN_POINT('Ctrl Pts',(-20.8309456072997,18.9176173210361,
-4.69152884528225));
#109172=CARTESIAN_POINT('Ctrl Pts',(-20.8360618081696,18.9568542469709,
-4.69377781537916));
#109173=CARTESIAN_POINT('Ctrl Pts',(-20.8416060197797,19.0112165349641,
-4.69695246402515));
#109174=CARTESIAN_POINT('Ctrl Pts',(-20.8429760800736,19.026239521453,-4.69783594811567));
#109175=CARTESIAN_POINT('Ctrl Pts',(-20.8450676744916,19.0522443113994,
-4.69937788773868));
#109176=CARTESIAN_POINT('Ctrl Pts',(-20.8458643545381,19.0632196518257,
-4.70003254732585));
#109177=CARTESIAN_POINT('Ctrl Pts',(-20.8468897380146,19.0790544973032,
-4.70098330192273));
#109178=CARTESIAN_POINT('Ctrl Pts',(-20.8471873277636,19.0839095700263,
-4.70127565419431));
#109179=CARTESIAN_POINT('Ctrl Pts',(-20.8476764825879,19.0923671965251,
-4.70178647414755));
#109180=CARTESIAN_POINT('Ctrl Pts',(-20.84787557773,19.0959693221584,-4.70200452015391));
#109181=CARTESIAN_POINT('Ctrl Pts',(-20.8482735902895,19.1035206038077,
-4.70246266329076));
#109182=CARTESIAN_POINT('Ctrl Pts',(-20.8484706505092,19.1074697979176,
-4.70270285852817));
#109183=CARTESIAN_POINT('Ctrl Pts',(-20.848964202122,19.1179506854619,-4.70334185429437));
#109184=CARTESIAN_POINT('Ctrl Pts',(-20.8492414964507,19.1244831790916,
-4.70374170623453));
#109185=CARTESIAN_POINT('Ctrl Pts',(-20.8502933314094,19.1523033146856,
-4.70545099609565));
#109186=CARTESIAN_POINT('Ctrl Pts',(-20.8507767753185,19.1735998854538,
-4.70677548760904));
#109187=CARTESIAN_POINT('Ctrl Pts',(-20.8509781232032,19.2000731000563,
-4.70843884822058));
#109188=CARTESIAN_POINT('Ctrl Pts',(-20.8509985064406,19.2052471210507,
-4.70876474515027));
#109189=CARTESIAN_POINT('Ctrl Pts',(-20.8510131828851,19.2589278683963,
-4.7121539328038));
#109190=CARTESIAN_POINT('Ctrl Pts',(-20.8493592891371,19.3074176151465,
-4.71528277626609));
#109191=CARTESIAN_POINT('Ctrl Pts',(-20.832613865767,19.5516578066844,-4.73125348668508));
#109192=CARTESIAN_POINT('Ctrl Pts',(-20.7920024870032,19.7447399655909,
-4.74444612677021));
#109193=CARTESIAN_POINT('Ctrl Pts',(-20.7092042732007,19.9742315272296,
-4.75978162116536));
#109194=CARTESIAN_POINT('Ctrl Pts',(-20.6915455002663,20.018446884523,-4.7627264078559));
#109195=CARTESIAN_POINT('Ctrl Pts',(-20.6673796319026,20.0734898719441,
-4.76638235984744));
#109196=CARTESIAN_POINT('Ctrl Pts',(-20.662247765335,20.0849028242802,-4.76713988539493));
#109197=CARTESIAN_POINT('Ctrl Pts',(-20.6539422341594,20.1029443980147,
-4.76833671410158));
#109198=CARTESIAN_POINT('Ctrl Pts',(-20.6508347893938,20.1096030179948,
-4.7687782839561));
#109199=CARTESIAN_POINT('Ctrl Pts',(-20.6449719433175,20.121997100207,-4.76959998081871));
#109200=CARTESIAN_POINT('Ctrl Pts',(-20.6422252384812,20.1277365626624,
-4.76998040307929));
#109201=CARTESIAN_POINT('Ctrl Pts',(-20.6360566866592,20.1404784025923,
-4.77082479695357));
#109202=CARTESIAN_POINT('Ctrl Pts',(-20.6326219523546,20.1474744655748,
-4.77128831416521));
#109203=CARTESIAN_POINT('Ctrl Pts',(-20.6224963103992,20.1678142466625,
-4.77263570211444));
#109204=CARTESIAN_POINT('Ctrl Pts',(-20.6157027253359,20.1811065341187,
-4.77351597527304));
#109205=CARTESIAN_POINT('Ctrl Pts',(-20.558759768144,20.2896716260239,-4.78070600382613));
#109206=CARTESIAN_POINT('Ctrl Pts',(-20.5015469788767,20.3810695699785,
-4.78674995809186));
#109207=CARTESIAN_POINT('Ctrl Pts',(-20.3582447177962,20.575330257831,-4.80001594074904));
#109208=CARTESIAN_POINT('Ctrl Pts',(-20.2688570844537,20.6751648623422,
-4.80713493129164));
#109209=CARTESIAN_POINT('Ctrl Pts',(-20.1586027802066,20.7770348723684,
-4.81548102759713));
#109210=CARTESIAN_POINT('Ctrl Pts',(-20.1464207329849,20.7880307404332,
-4.81639816825224));
#109211=CARTESIAN_POINT('Ctrl Pts',(-20.0943095302242,20.8339796585553,
-4.82030630858372));
#109212=CARTESIAN_POINT('Ctrl Pts',(-20.0532046867677,20.8675636056931,
-4.82335191687341));
#109213=CARTESIAN_POINT('Ctrl Pts',(-20.003943197236,20.9048149355989,-4.82701708480235));
#109214=CARTESIAN_POINT('Ctrl Pts',(-19.9969684920759,20.9100218781408,
-4.82753636384703));
#109215=CARTESIAN_POINT('Ctrl Pts',(-19.9863558179364,20.9178432773327,
-4.82832734833898));
#109216=CARTESIAN_POINT('Ctrl Pts',(-19.982741235141,20.9204895129556,-4.82859689903229));
#109217=CARTESIAN_POINT('Ctrl Pts',(-19.9762361354366,20.9252202554302,
-4.82908232405857));
#109218=CARTESIAN_POINT('Ctrl Pts',(-19.9733487323991,20.9273089522324,
-4.82929790348169));
#109219=CARTESIAN_POINT('Ctrl Pts',(-19.9670610085826,20.9318332408804,
-4.82976761890079));
#109220=CARTESIAN_POINT('Ctrl Pts',(-19.9636587841079,20.9342660177041,
-4.83002193712546));
#109221=CARTESIAN_POINT('Ctrl Pts',(-19.9540761796022,20.9410752778455,
-4.83073863844566));
#109222=CARTESIAN_POINT('Ctrl Pts',(-19.9478795653868,20.9454286516895,
-4.83120255612889));
#109223=CARTESIAN_POINT('Ctrl Pts',(-19.9105753596477,20.9713385450178,
-4.83399748170086));
#109224=CARTESIAN_POINT('Ctrl Pts',(-19.8789196688878,20.9920895292447,
-4.83637782586188));
#109225=CARTESIAN_POINT('Ctrl Pts',(-19.7726333764,21.0577580499199,-4.84435459582894));
#109226=CARTESIAN_POINT('Ctrl Pts',(-19.6957896019241,21.0989177493281,
-4.85009413751182));
#109227=CARTESIAN_POINT('Ctrl Pts',(-19.4572820078323,21.2083203148315,
-4.8674314078552));
#109228=CARTESIAN_POINT('Ctrl Pts',(-19.2894325710295,21.2613520087403,
-4.878941108188));
#109229=CARTESIAN_POINT('Ctrl Pts',(-19.0943196570524,21.2972377133742,
-4.89115222507541));
#109230=CARTESIAN_POINT('Ctrl Pts',(-19.071630994555,21.3010295282562,-4.8925563738403));
#109231=CARTESIAN_POINT('Ctrl Pts',(-19.0394427402428,21.3058710921219,
-4.89452680396895));
#109232=CARTESIAN_POINT('Ctrl Pts',(-19.0299915462981,21.3072273658568,
-4.89510274391011));
#109233=CARTESIAN_POINT('Ctrl Pts',(-19.0146191859176,21.3093273049685,
-4.89603533532351));
#109234=CARTESIAN_POINT('Ctrl Pts',(-19.0087035597605,21.3101099451123,
-4.89639321500522));
#109235=CARTESIAN_POINT('Ctrl Pts',(-18.9963132097617,21.3116959193959,
-4.89714073136632));
#109236=CARTESIAN_POINT('Ctrl Pts',(-18.9898379136981,21.3124943562061,
-4.8975302096955));
#109237=CARTESIAN_POINT('Ctrl Pts',(-18.9744233690518,21.314322745566,-4.89845461297006));
#109238=CARTESIAN_POINT('Ctrl Pts',(-18.9654809949011,21.3153256689991,
-4.89898868062658));
#109239=CARTESIAN_POINT('Ctrl Pts',(-18.9353272527073,21.3185129938539,
-4.90078234748879));
#109240=CARTESIAN_POINT('Ctrl Pts',(-18.9140889178629,21.3204339791789,
-4.90203366321955));
#109241=CARTESIAN_POINT('Ctrl Pts',(-18.7982761315433,21.3291472072138,
-4.90879695704966));
#109242=CARTESIAN_POINT('Ctrl Pts',(-18.7033508508947,21.3299012893246,
-4.91411575375226));
#109243=CARTESIAN_POINT('Ctrl Pts',(-18.4395215028324,21.3142566389095,
-4.92865780770001));
#109244=CARTESIAN_POINT('Ctrl Pts',(-18.2721941620099,21.2839519864042,
-4.93757509024029));
#109245=CARTESIAN_POINT('Ctrl Pts',(-18.0737538983856,21.2227717633758,
-4.94941814878349));
#109246=CARTESIAN_POINT('Ctrl Pts',(-18.0375349713775,21.210521592313,-4.951636370292));
#109247=CARTESIAN_POINT('Ctrl Pts',(-17.9948878103104,21.1947979796451,
-4.95433812312448));
#109248=CARTESIAN_POINT('Ctrl Pts',(-17.9881184371085,21.1922627144682,
-4.95476970105525));
#109249=CARTESIAN_POINT('Ctrl Pts',(-17.9771200668849,21.1880792515937,
-4.95547555231606));
#109250=CARTESIAN_POINT('Ctrl Pts',(-17.9728830883416,21.1864520105893,
-4.95574860210258));
#109251=CARTESIAN_POINT('Ctrl Pts',(-17.9653246456289,21.1835212118046,
-4.95623777778179));
#109252=CARTESIAN_POINT('Ctrl Pts',(-17.9620012144587,21.1822228707841,
-4.95645358885821));
#109253=CARTESIAN_POINT('Ctrl Pts',(-17.9548296228134,21.1794002780123,
-4.95692085923091));
#109254=CARTESIAN_POINT('Ctrl Pts',(-17.9509826995798,21.1778731625931,
-4.95717248481111));
#109255=CARTESIAN_POINT('Ctrl Pts',(-17.940295425491,21.173594306322,-4.9578742035031));
#109256=CARTESIAN_POINT('Ctrl Pts',(-17.9334650121597,21.17081812737,-4.95832573192174));
#109257=CARTESIAN_POINT('Ctrl Pts',(-17.8947278876086,21.1548373708101,
-4.96090325753113));
#109258=CARTESIAN_POINT('Ctrl Pts',(-17.8631354718184,21.1408901674283,
-4.96307025179287));
#109259=CARTESIAN_POINT('Ctrl Pts',(-17.7643048239258,21.0943383068067,
-4.97002488772784));
#109260=CARTESIAN_POINT('Ctrl Pts',(-17.6984466828193,21.0589447247882,
-4.97492054677147));
#109261=CARTESIAN_POINT('Ctrl Pts',(-17.4687641306777,20.9193692854144,
-4.99264725939744));
#109262=CARTESIAN_POINT('Ctrl Pts',(-17.3175289671192,20.7962409338101,
-5.00547118345634));
#109263=CARTESIAN_POINT('Ctrl Pts',(-17.1707717429345,20.6387440610431,
-5.01869701004288));
#109264=CARTESIAN_POINT('Ctrl Pts',(-17.1565955201768,20.6230661618369,
-5.01998563759317));
#109265=CARTESIAN_POINT('Ctrl Pts',(-17.1371815480636,20.6009383928977,
-5.02176659476284));
#109266=CARTESIAN_POINT('Ctrl Pts',(-17.1317437440633,20.594666433024,-5.02226726499616));
#109267=CARTESIAN_POINT('Ctrl Pts',(-17.1224153529102,20.5837783383507,
-5.02312938811789));
#109268=CARTESIAN_POINT('Ctrl Pts',(-17.1185073911103,20.5791772811945,
-5.02349155747948));
#109269=CARTESIAN_POINT('Ctrl Pts',(-17.110450064857,20.5696082967367,-5.02424037796577));
#109270=CARTESIAN_POINT('Ctrl Pts',(-17.1063036925789,20.5646379235632,
-5.02462690412941));
#109271=CARTESIAN_POINT('Ctrl Pts',(-17.096636871529,20.5529413920255,-5.02553086844356));
#109272=CARTESIAN_POINT('Ctrl Pts',(-17.09113494064,20.5462000278192,-5.02604755105093));
#109273=CARTESIAN_POINT('Ctrl Pts',(-17.0733642628319,20.5241499597974,
-5.02772372748138));
#109274=CARTESIAN_POINT('Ctrl Pts',(-17.0612664883158,20.5087043213395,
-5.0288763675597));
#109275=CARTESIAN_POINT('Ctrl Pts',(-17.0002432388907,20.4285223517193,
-5.03475463679033));
#109276=CARTESIAN_POINT('Ctrl Pts',(-16.9548515451049,20.3611765254235,
-5.03934111643026));
#109277=CARTESIAN_POINT('Ctrl Pts',(-16.8273869862402,20.1463849159155,
-5.0531834560534));
#109278=CARTESIAN_POINT('Ctrl Pts',(-16.7589776858456,19.9916389950774,
-5.06205516023817));
#109279=CARTESIAN_POINT('Ctrl Pts',(-16.6938951184651,19.778943811717,-5.07455912022939));
#109280=CARTESIAN_POINT('Ctrl Pts',(-16.6801120430088,19.726879167981,-5.07764762117836));
#109281=CARTESIAN_POINT('Ctrl Pts',(-16.6664168246377,19.6658243312195,
-5.08136069197208));
#109282=CARTESIAN_POINT('Ctrl Pts',(-16.6645570906476,19.6572862291036,
-5.08188199393419));
#109283=CARTESIAN_POINT('Ctrl Pts',(-16.6618224896651,19.6443468588404,
-5.08267546015003));
#109284=CARTESIAN_POINT('Ctrl Pts',(-16.6609086438301,19.6399537999906,
-5.08294544936315));
#109285=CARTESIAN_POINT('Ctrl Pts',(-16.6592939844144,19.6320660906188,
-5.08343134068244));
#109286=CARTESIAN_POINT('Ctrl Pts',(-16.6585880239935,19.6285725485843,
-5.08364694537929));
#109287=CARTESIAN_POINT('Ctrl Pts',(-16.6570738986891,19.6209809947263,
-5.08411633735494));
#109288=CARTESIAN_POINT('Ctrl Pts',(-16.6562690491018,19.6168824230329,
-5.08437030479705));
#109289=CARTESIAN_POINT('Ctrl Pts',(-16.6540440284857,19.6053717945954,
-5.08508504842686));
#109290=CARTESIAN_POINT('Ctrl Pts',(-16.6526513722592,19.5979545731375,
-5.08554734605958));
#109291=CARTESIAN_POINT('Ctrl Pts',(-16.6445949017933,19.5537440623794,
-5.08831253120777));
#109292=CARTESIAN_POINT('Ctrl Pts',(-16.6388676284481,19.5167893152632,
-5.09066356707414));
#109293=CARTESIAN_POINT('Ctrl Pts',(-16.6232937521079,19.3950825083755,
-5.09849443678796));
#109294=CARTESIAN_POINT('Ctrl Pts',(-16.6175911268477,19.3098880430378,
-5.10411213130873));
#109295=CARTESIAN_POINT('Ctrl Pts',(-16.6159018569454,19.0467103331915,
-5.12149861875124));
#109296=CARTESIAN_POINT('Ctrl Pts',(-16.6371840536535,18.8693596482302,
-5.13318742502556));
#109297=CARTESIAN_POINT('Ctrl Pts',(-16.6859509173027,18.6746195928484,
-5.14554188538172));
#109298=CARTESIAN_POINT('Ctrl Pts',(-16.6918474567328,18.6525897205716,
-5.14693377490617));
#109299=CARTESIAN_POINT('Ctrl Pts',(-16.7007074227669,18.6215079853256,
-5.14889014403152));
#109300=CARTESIAN_POINT('Ctrl Pts',(-16.7033775721471,18.6123748250191,
-5.14946409630717));
#109301=CARTESIAN_POINT('Ctrl Pts',(-16.7078205653842,18.5975495661295,
-5.15039434856947));
#109302=CARTESIAN_POINT('Ctrl Pts',(-16.7095560126518,18.5918464816418,
-5.15075186458501));
#109303=CARTESIAN_POINT('Ctrl Pts',(-16.7132427569742,18.5799122102266,
-5.15149931912294));
#109304=CARTESIAN_POINT('Ctrl Pts',(-16.7151988422498,18.5736825590166,
-5.15188909623111));
#109305=CARTESIAN_POINT('Ctrl Pts',(-16.7199277478882,18.5588624025487,
-5.15281547913382));
#109306=CARTESIAN_POINT('Ctrl Pts',(-16.7227267666955,18.550280341164,-5.15335121773151));
#109307=CARTESIAN_POINT('Ctrl Pts',(-16.7323753618707,18.5213263613745,
-5.15515647736733));
#109308=CARTESIAN_POINT('Ctrl Pts',(-16.7394803852505,18.501040510862,-5.15641756600282));
#109309=CARTESIAN_POINT('Ctrl Pts',(-16.8087628236532,18.3124839420369,
-5.16811368785506));
#109310=CARTESIAN_POINT('Ctrl Pts',(-16.8917804855617,18.152650556414,-5.1777525891409));
#109311=CARTESIAN_POINT('Ctrl Pts',(-17.0626408164904,17.9060925369895,
-5.1940778535634));
#109312=CARTESIAN_POINT('Ctrl Pts',(-17.1396434648458,17.8130573118082,
-5.20069209329022));
#109313=CARTESIAN_POINT('Ctrl Pts',(-17.2307836023472,17.7203224366964,
-5.2083981773159));
#109314=CARTESIAN_POINT('Ctrl Pts',(-17.2374837298306,17.71359618625,-5.20896408525885));
#109315=CARTESIAN_POINT('Ctrl Pts',(-17.2474829264602,17.7036921452285,
-5.20980817647847));
#109316=CARTESIAN_POINT('Ctrl Pts',(-17.2507475386143,17.7004795221945,
-5.21008368936304));
#109317=CARTESIAN_POINT('Ctrl Pts',(-17.256576471903,17.6947805315728,-5.2105755435686));
#109318=CARTESIAN_POINT('Ctrl Pts',(-17.2591366849665,17.6922900344208,
-5.21079155609991));
#109319=CARTESIAN_POINT('Ctrl Pts',(-17.2646568836004,17.6869472769438,
-5.2112572794998));
#109320=CARTESIAN_POINT('Ctrl Pts',(-17.2676188337563,17.6840971966141,
-5.21150714611296));
#109321=CARTESIAN_POINT('Ctrl Pts',(-17.2758230784177,17.6762487069792,
-5.21219912973855));
#109322=CARTESIAN_POINT('Ctrl Pts',(-17.281082697005,17.671268603545,-5.21264261914473));
#109323=CARTESIAN_POINT('Ctrl Pts',(-17.310127522781,17.6440486546061,-5.21509042629719));
#109324=CARTESIAN_POINT('Ctrl Pts',(-17.33439648886,17.6223341786083,-5.21713114492648));
#109325=CARTESIAN_POINT('Ctrl Pts',(-17.4828610820487,17.4955392507688,
-5.2295377243308));
#109326=CARTESIAN_POINT('Ctrl Pts',(-17.6183289249666,17.4045027926796,
-5.24049306500456));
#109327=CARTESIAN_POINT('Ctrl Pts',(-17.8667114725002,17.2762770854998,
-5.25875157455107));
#109328=CARTESIAN_POINT('Ctrl Pts',(-17.9748111309381,17.2313580573907,
-5.2661945320723));
#109329=CARTESIAN_POINT('Ctrl Pts',(-18.0996627134878,17.1912206345028,
-5.27420196279347));
#109330=CARTESIAN_POINT('Ctrl Pts',(-18.1132868275275,17.1869921809681,
-5.27506841447953));
#109331=CARTESIAN_POINT('Ctrl Pts',(-18.1350455017289,17.1804794099915,
-5.27644077317913));
#109332=CARTESIAN_POINT('Ctrl Pts',(-18.1431526121031,17.1781055795014,
-5.27694959534783));
#109333=CARTESIAN_POINT('Ctrl Pts',(-18.1574799708308,17.1740033554253,
-5.27784446364162));
#109334=CARTESIAN_POINT('Ctrl Pts',(-18.1636942828096,17.1722547818784,
-5.27823116354203));
#109335=CARTESIAN_POINT('Ctrl Pts',(-18.1765680460805,17.1686958501921,
-5.27902933029003));
#109336=CARTESIAN_POINT('Ctrl Pts',(-18.1832285533561,17.1668895727313,
-5.27944066052309));
#109337=CARTESIAN_POINT('Ctrl Pts',(-18.2003562700842,17.1623344624698,
-5.28049432529007));
#109338=CARTESIAN_POINT('Ctrl Pts',(-18.2108360221574,17.1596332424422,
-5.281135113029));
#109339=CARTESIAN_POINT('Ctrl Pts',(-18.2547329082635,17.1486768247096,
-5.28380335969078));
#109340=CARTESIAN_POINT('Ctrl Pts',(-18.2883292540094,17.1411566220439,
-5.28580711839118));
#109341=CARTESIAN_POINT('Ctrl Pts',(-18.3763995201453,17.1236869300678,
-5.2909721489968));
#109342=CARTESIAN_POINT('Ctrl Pts',(-18.4311076203829,17.1150489474822,
-5.29409360975679));
#109343=CARTESIAN_POINT('Ctrl Pts',(-18.5949003264753,17.0957355807034,
-5.30326226489374));
#109344=CARTESIAN_POINT('Ctrl Pts',(-18.7045407716048,17.091371425147,-5.30916081290938));
#109345=CARTESIAN_POINT('Ctrl Pts',(-18.8742915571145,17.0977928571337,
-5.31841054153964));
#109346=CARTESIAN_POINT('Ctrl Pts',(-18.9344296986124,17.1026467482511,
-5.32171287893654));
#109347=CARTESIAN_POINT('Ctrl Pts',(-19.0521169367126,17.1172264727426,
-5.32835560136133));
#109348=CARTESIAN_POINT('Ctrl Pts',(-19.1096323309069,17.126777116787,-5.33168831918916));
#109349=CARTESIAN_POINT('Ctrl Pts',(-19.1753930486656,17.1405071843618,
-5.3356734271783));
#109350=CARTESIAN_POINT('Ctrl Pts',(-19.184099648586,17.1423824367301,-5.33620462067294));
#109351=CARTESIAN_POINT('Ctrl Pts',(-19.1972096009958,17.1452927787057,
-5.33701021233555));
#109352=CARTESIAN_POINT('Ctrl Pts',(-19.2016220191159,17.1462871616305,
-5.33728233499326));
#109353=CARTESIAN_POINT('Ctrl Pts',(-19.2095082259081,17.1480909740058,
-5.33777051039889));
#109354=CARTESIAN_POINT('Ctrl Pts',(-19.2129831854314,17.1488950486842,
-5.33798625359744));
#109355=CARTESIAN_POINT('Ctrl Pts',(-19.2204970850207,17.1506537159885,
-5.33845414236567));
#109356=CARTESIAN_POINT('Ctrl Pts',(-19.2245351991588,17.1516113913403,
-5.33870645832793));
#109357=CARTESIAN_POINT('Ctrl Pts',(-19.2357892121002,17.1543153606621,
-5.33941200890397));
#109358=CARTESIAN_POINT('Ctrl Pts',(-19.2429986971229,17.1560877289673,
-5.33986670393191));
#109359=CARTESIAN_POINT('Ctrl Pts',(-19.2844761458584,17.1665161440709,
-5.34249767490051));
#109360=CARTESIAN_POINT('Ctrl Pts',(-19.3185302414702,17.1759908398913,
-5.34471692407298));
#109361=CARTESIAN_POINT('Ctrl Pts',(-19.4265704926763,17.2089857628015,
-5.35191368388791));
#109362=CARTESIAN_POINT('Ctrl Pts',(-19.4995040794923,17.2357236234289,
-5.357007154015));
#109363=CARTESIAN_POINT('Ctrl Pts',(-19.7408833899257,17.3395940313429,
-5.37434910975497));
#109364=CARTESIAN_POINT('Ctrl Pts',(-19.9006689751638,17.434800452723,-5.3865722435985));
#109365=CARTESIAN_POINT('Ctrl Pts',(-20.0654595660431,17.5649390226409,
-5.39951917268111));
#109366=CARTESIAN_POINT('Ctrl Pts',(-20.0846094189555,17.5806148933025,
-5.40103147641083));
#109367=CARTESIAN_POINT('Ctrl Pts',(-20.1109857464919,17.6029900146471,
-5.40312631445175));
#109368=CARTESIAN_POINT('Ctrl Pts',(-20.1184464140189,17.6094089189606,
-5.40372021400209));
#109369=CARTESIAN_POINT('Ctrl Pts',(-20.1303991086684,17.6198385419045,
-5.4046739996304));
#109370=CARTESIAN_POINT('Ctrl Pts',(-20.1349191947848,17.6238167505714,
-5.40503522572458));
#109371=CARTESIAN_POINT('Ctrl Pts',(-20.1439745301161,17.6318553334297,
-5.40576000532202));
#109372=CARTESIAN_POINT('Ctrl Pts',(-20.148509362761,17.6359160919527,-5.40612353770611));
#109373=CARTESIAN_POINT('Ctrl Pts',(-20.1592223937094,17.645592757452,-5.40698373637908));
#109374=CARTESIAN_POINT('Ctrl Pts',(-20.1653850385675,17.651225791672,-5.40747967371305));
#109375=CARTESIAN_POINT('Ctrl Pts',(-20.1845723145197,17.6689736185084,
-5.40902740829496));
#109376=CARTESIAN_POINT('Ctrl Pts',(-20.1974778979819,17.681216397125,-5.41007373642303));
#109377=CARTESIAN_POINT('Ctrl Pts',(-20.2271757093824,17.7101088026172,
-5.41249526894861));
#109378=CARTESIAN_POINT('Ctrl Pts',(-20.243846498808,17.7268801603108,-5.41386514614617));
#109379=CARTESIAN_POINT('Ctrl Pts',(-20.3005066310864,17.7858251661314,
-5.41856358981311));
#109380=CARTESIAN_POINT('Ctrl Pts',(-20.3390395385547,17.829365044568,-5.42183366041554));
#109381=CARTESIAN_POINT('Ctrl Pts',(-20.4797765659393,18.0022360320717,
-5.43419924150301));
#109382=CARTESIAN_POINT('Ctrl Pts',(-20.5685325627749,18.1417338121171,
-5.44288447751858));
#109383=CARTESIAN_POINT('Ctrl Pts',(-20.6659521660254,18.3433873181785,
-5.4554206781514));
#109384=CARTESIAN_POINT('Ctrl Pts',(-20.689446336058,18.3977231612727,-5.45880237458842));
#109385=CARTESIAN_POINT('Ctrl Pts',(-20.713832068521,18.4613108250018,-5.46284207578789));
#109386=CARTESIAN_POINT('Ctrl Pts',(-20.716979372528,18.4696757251889,-5.46337510271013));
#109387=CARTESIAN_POINT('Ctrl Pts',(-20.7209131560224,18.4803352400332,
-5.46405668761308));
#109388=CARTESIAN_POINT('Ctrl Pts',(-20.7217488443111,18.4826117705353,
-5.46420238754676));
#109389=CARTESIAN_POINT('Ctrl Pts',(-20.7225806137986,18.4848897174502,
-5.46434831804488));
#109390=CARTESIAN_POINT('Ctrl Pts',(-20.7225806829213,18.4848899067551,
-5.24452709861031));
#109391=CARTESIAN_POINT('Ctrl Pts',(-20.7014125433041,18.4269172192414,
-5.24117488823769));
#109392=CARTESIAN_POINT('Ctrl Pts',(-20.6777012897646,18.3698481845845,
-5.23782825408735));
#109393=CARTESIAN_POINT('Ctrl Pts',(-20.6249328374919,18.2570646671581,
-5.23098491305862));
#109394=CARTESIAN_POINT('Ctrl Pts',(-20.5958563006109,18.2014904246063,
-5.22749307031487));
#109395=CARTESIAN_POINT('Ctrl Pts',(-20.5488220101447,18.1205568429588,
-5.22210871730596));
#109396=CARTESIAN_POINT('Ctrl Pts',(-20.5327016390253,18.0941663534545,
-5.22030291401821));
#109397=CARTESIAN_POINT('Ctrl Pts',(-20.5121619838508,18.0621397956072,
-5.21803698818975));
#109398=CARTESIAN_POINT('Ctrl Pts',(-20.5082836603195,18.0561591886834,
-5.21761058962982));
#109399=CARTESIAN_POINT('Ctrl Pts',(-20.5021352906482,18.0467821156106,
-5.21693669652013));
#109400=CARTESIAN_POINT('Ctrl Pts',(-20.4998854489977,18.0433723758248,
-5.21669053392754));
#109401=CARTESIAN_POINT('Ctrl Pts',(-20.4956478283958,18.0369903259839,
-5.2162276453178));
#109402=CARTESIAN_POINT('Ctrl Pts',(-20.4936623833455,18.0340165328543,
-5.21601107548901));
#109403=CARTESIAN_POINT('Ctrl Pts',(-20.4890946288609,18.0272123569264,
-5.215513541008));
#109404=CARTESIAN_POINT('Ctrl Pts',(-20.4865073169418,18.0233853978325,
-5.21523224147417));
#109405=CARTESIAN_POINT('Ctrl Pts',(-20.478451206119,18.0115530507845,-5.21435803667393));
#109406=CARTESIAN_POINT('Ctrl Pts',(-20.47294001505,18.0035768718607,-5.21376236557274));
#109407=CARTESIAN_POINT('Ctrl Pts',(-20.4106715053545,17.9147681654412,
-5.20706098688228));
#109408=CARTESIAN_POINT('Ctrl Pts',(-20.3483849544847,17.8379738181674,
-5.20062772543763));
#109409=CARTESIAN_POINT('Ctrl Pts',(-20.1664593538686,17.643234191429,-5.18307327694679));
#109410=CARTESIAN_POINT('Ctrl Pts',(-20.0377574008985,17.5346758714274,
-5.17192757325268));
#109411=CARTESIAN_POINT('Ctrl Pts',(-19.8712093636095,17.425099666453,-5.15940141897003));
#109412=CARTESIAN_POINT('Ctrl Pts',(-19.8444569313007,17.408343430679,-5.15743879867111));
#109413=CARTESIAN_POINT('Ctrl Pts',(-19.8041717225822,17.3843483202024,
-5.1545552746295));
#109414=CARTESIAN_POINT('Ctrl Pts',(-19.7909197488194,17.3766487416391,
-5.15361796646791));
#109415=CARTESIAN_POINT('Ctrl Pts',(-19.7666473255767,17.3628965021666,
-5.15192126657722));
#109416=CARTESIAN_POINT('Ctrl Pts',(-19.7556544359079,17.3567968660354,
-5.15116021287474));
#109417=CARTESIAN_POINT('Ctrl Pts',(-19.7382624489895,17.3473481873539,
-5.14996752839326));
#109418=CARTESIAN_POINT('Ctrl Pts',(-19.7318995657547,17.343933422744,-5.14953355739942));
#109419=CARTESIAN_POINT('Ctrl Pts',(-19.7254731426295,17.3405267951213,
-5.14909761334312));
#109420=CARTESIAN_POINT('Ctrl Pts',(-19.7254270105499,17.3405023428304,
-5.14909448404078));
#109421=CARTESIAN_POINT('Ctrl Pts',(-19.7253331203011,17.3404525807897,
-5.14908811538135));
#109422=CARTESIAN_POINT('Ctrl Pts',(-19.7252853611042,17.3404272706519,
-5.14908487596325));
#109423=CARTESIAN_POINT('Ctrl Pts',(-19.7251881573754,17.3403757619958,
-5.14907828308036));
#109424=CARTESIAN_POINT('Ctrl Pts',(-19.7251387117589,17.3403495630709,
-5.14907492955136));
#109425=CARTESIAN_POINT('Ctrl Pts',(-19.7250380735856,17.3402962447093,
-5.1490681042969));
#109426=CARTESIAN_POINT('Ctrl Pts',(-19.7249868802129,17.3402691250206,
-5.14906463252616));
#109427=CARTESIAN_POINT('Ctrl Pts',(-19.7248826827138,17.340213931874,-5.14905756649119));
#109428=CARTESIAN_POINT('Ctrl Pts',(-19.7248296777858,17.3401858581848,
-5.14905397218336));
#109429=CARTESIAN_POINT('Ctrl Pts',(-19.7247217910763,17.3401287226155,
-5.14904665662473));
#109430=CARTESIAN_POINT('Ctrl Pts',(-19.7246669085466,17.3400996605466,
-5.14904293533475));
#109431=CARTESIAN_POINT('Ctrl Pts',(-19.7245551981646,17.3400405125918,
-5.14903536120447));
#109432=CARTESIAN_POINT('Ctrl Pts',(-19.724498369524,17.340010426511,-5.14903150832312));
#109433=CARTESIAN_POINT('Ctrl Pts',(-19.7243826959561,17.3399491936393,
-5.14902366623662));
#109434=CARTESIAN_POINT('Ctrl Pts',(-19.7243238502478,17.3399180466738,
-5.14901967699182));
#109435=CARTESIAN_POINT('Ctrl Pts',(-19.7242040688028,17.3398546537271,
-5.14901155721985));
#109436=CARTESIAN_POINT('Ctrl Pts',(-19.724143132582,17.3398224077461,-5.14900742667415));
#109437=CARTESIAN_POINT('Ctrl Pts',(-19.7240190939745,17.3397567772569,
-5.14899901918283));
#109438=CARTESIAN_POINT('Ctrl Pts',(-19.7239559908874,17.3397233926534,
-5.14899474220509));
#109439=CARTESIAN_POINT('Ctrl Pts',(-19.7238275395831,17.3396554439795,
-5.14898603654433));
#109440=CARTESIAN_POINT('Ctrl Pts',(-19.7237621908733,17.3396208799438,
-5.14898160784439));
#109441=CARTESIAN_POINT('Ctrl Pts',(-19.7236291644548,17.3395505289426,
-5.14897259310541));
#109442=CARTESIAN_POINT('Ctrl Pts',(-19.7235614894262,17.3395147437117,
-5.14896800726576));
#109443=CARTESIAN_POINT('Ctrl Pts',(-19.7234348804973,17.3394478041748,
-5.1489594283989));
#109444=CARTESIAN_POINT('Ctrl Pts',(-19.7233759456494,17.3394166482323,
-5.14895543524413));
#109445=CARTESIAN_POINT('Ctrl Pts',(-19.7232483249391,17.3393491891808,
-5.14894678868114));
#109446=CARTESIAN_POINT('Ctrl Pts',(-19.7231796374951,17.3393128865111,
-5.14894213523691));
#109447=CARTESIAN_POINT('Ctrl Pts',(-19.7230309151709,17.3392342943013,
-5.14893206016565));
#109448=CARTESIAN_POINT('Ctrl Pts',(-19.7229508786399,17.3391920056183,
-5.14892663852325));
#109449=CARTESIAN_POINT('Ctrl Pts',(-19.7227776081786,17.3391004693942,
-5.1489149020452));
#109450=CARTESIAN_POINT('Ctrl Pts',(-19.7226843726364,17.3390512233444,
-5.14890858723104));
#109451=CARTESIAN_POINT('Ctrl Pts',(-19.722482564125,17.3389446494573,-5.14889491987937));
#109452=CARTESIAN_POINT('Ctrl Pts',(-19.7223739893192,17.3388873238205,
-5.14888756739431));
#109453=CARTESIAN_POINT('Ctrl Pts',(-19.722139031633,17.3387632963257,-5.1488716579522));
#109454=CARTESIAN_POINT('Ctrl Pts',(-19.7220126472998,17.3386965979849,
-5.14886310113573));
#109455=CARTESIAN_POINT('Ctrl Pts',(-19.7217267234242,17.338545740914,-5.14884374480244));
#109456=CARTESIAN_POINT('Ctrl Pts',(-19.7215671798329,17.3384615897524,
-5.14883294555272));
#109457=CARTESIAN_POINT('Ctrl Pts',(-19.7156957213096,17.3353656519479,
-5.14843556941465));
#109458=CARTESIAN_POINT('Ctrl Pts',(-19.7099700189701,17.3323799691455,
-5.14804992011967));
#109459=CARTESIAN_POINT('Ctrl Pts',(-19.696713171875,17.3255441165983,-5.14716126293205));
#109460=CARTESIAN_POINT('Ctrl Pts',(-19.6891724024991,17.3217127734971,
-5.14665892224424));
#109461=CARTESIAN_POINT('Ctrl Pts',(-19.6688198146561,17.3115249530066,
-5.14531140744099));
#109462=CARTESIAN_POINT('Ctrl Pts',(-19.6559660706415,17.3052528710352,
-5.14446918099384));
#109463=CARTESIAN_POINT('Ctrl Pts',(-19.5375059312837,17.2489283902529,
-5.13678499774756));
#109464=CARTESIAN_POINT('Ctrl Pts',(-19.4279819250668,17.207567661172,-5.13025988143086));
#109465=CARTESIAN_POINT('Ctrl Pts',(-19.1589193143186,17.1306918040814,
-5.1149410087118));
#109466=CARTESIAN_POINT('Ctrl Pts',(-18.9976237312764,17.1041708180831,
-5.10633095074161));
#109467=CARTESIAN_POINT('Ctrl Pts',(-18.8026648418282,17.0948676944578,
-5.09512111302561));
#109468=CARTESIAN_POINT('Ctrl Pts',(-18.7703956710023,17.0940668659299,
-5.09323823541426));
#109469=CARTESIAN_POINT('Ctrl Pts',(-18.7308991355655,17.0939899464402,
-5.09088648674902));
#109470=CARTESIAN_POINT('Ctrl Pts',(-18.723675515846,17.0940128522262,-5.09045443858482));
#109471=CARTESIAN_POINT('Ctrl Pts',(-18.7123462099846,17.0941067636048,
-5.08977360226996));
#109472=CARTESIAN_POINT('Ctrl Pts',(-18.7082402941069,17.0941527457534,
-5.0895261921682));
#109473=CARTESIAN_POINT('Ctrl Pts',(-18.7005624824496,17.0942610706968,
-5.08906226477376));
#109474=CARTESIAN_POINT('Ctrl Pts',(-18.6969906018764,17.0943205093357,
-5.08884591155034));
#109475=CARTESIAN_POINT('Ctrl Pts',(-18.6888329401159,17.0944769135551,
-5.08835060330778));
#109476=CARTESIAN_POINT('Ctrl Pts',(-18.6842473284257,17.094579741755,-5.08807132460394));
#109477=CARTESIAN_POINT('Ctrl Pts',(-18.6701380455842,17.0949420095614,
-5.08720946956608));
#109478=CARTESIAN_POINT('Ctrl Pts',(-18.6606159162784,17.0952508332552,
-5.0866242366605));
#109479=CARTESIAN_POINT('Ctrl Pts',(-18.5315791820128,17.1003079053782,
-5.07864800885465));
#109480=CARTESIAN_POINT('Ctrl Pts',(-18.4126873485253,17.1151119175829,
-5.07078011330997));
#109481=CARTESIAN_POINT('Ctrl Pts',(-18.1890882319371,17.1624310789412,
-5.05568137314921));
#109482=CARTESIAN_POINT('Ctrl Pts',(-18.0843720809438,17.1931916586331,
-5.04847842249467));
#109483=CARTESIAN_POINT('Ctrl Pts',(-17.9123334388415,17.2585185535274,
-5.03665456987097));
#109484=CARTESIAN_POINT('Ctrl Pts',(-17.843642548131,17.2888695436925,-5.0319334881336));
#109485=CARTESIAN_POINT('Ctrl Pts',(-17.7599263962632,17.3313129614492,
-5.02618353657497));
#109486=CARTESIAN_POINT('Ctrl Pts',(-17.743264689758,17.3400413341629,-5.02503916606737));
#109487=CARTESIAN_POINT('Ctrl Pts',(-17.7191970199992,17.3530610639241,
-5.02338572328093));
#109488=CARTESIAN_POINT('Ctrl Pts',(-17.7116976121879,17.357176920622,-5.02287045509809));
#109489=CARTESIAN_POINT('Ctrl Pts',(-17.6985884661601,17.3644752782391,
-5.02196958001907));
#109490=CARTESIAN_POINT('Ctrl Pts',(-17.6929679781688,17.3676381463661,
-5.02158327719278));
#109491=CARTESIAN_POINT('Ctrl Pts',(-17.6820791682244,17.3738313903971,
-5.02083472989412));
#109492=CARTESIAN_POINT('Ctrl Pts',(-17.6768092755527,17.3768588631839,
-5.0204723858907));
#109493=CARTESIAN_POINT('Ctrl Pts',(-17.6642373732314,17.3841534143028,
-5.01960777290718));
#109494=CARTESIAN_POINT('Ctrl Pts',(-17.6569477165769,17.3884416587577,
-5.01910627444909));
#109495=CARTESIAN_POINT('Ctrl Pts',(-17.6307061322636,17.4040910695468,
-5.01730018326313));
#109496=CARTESIAN_POINT('Ctrl Pts',(-17.6119062466824,17.4157053432614,
-5.01600481466161));
#109497=CARTESIAN_POINT('Ctrl Pts',(-17.4368626908648,17.527668504883,-5.0039196874903));
#109498=CARTESIAN_POINT('Ctrl Pts',(-17.2942816929144,17.6478661852732,
-4.99398766922138));
#109499=CARTESIAN_POINT('Ctrl Pts',(-17.115269924403,17.8443201817385,-4.97949851819132));
#109500=CARTESIAN_POINT('Ctrl Pts',(-17.0647433244534,17.9065150704033,
-4.97509479861646));
#109501=CARTESIAN_POINT('Ctrl Pts',(-16.996778301074,18.0006089018065,-4.96845519607244));
#109502=CARTESIAN_POINT('Ctrl Pts',(-16.9764418056879,18.0303329481552,
-4.96636050073923));
#109503=CARTESIAN_POINT('Ctrl Pts',(-16.9528178321274,18.0668257068903,
-4.96377343218186));
#109504=CARTESIAN_POINT('Ctrl Pts',(-16.9487943018253,18.0731136526,-4.96332712398541));
#109505=CARTESIAN_POINT('Ctrl Pts',(-16.9425810720058,18.0829377134332,
-4.96262877614957));
#109506=CARTESIAN_POINT('Ctrl Pts',(-16.9403683486528,18.086459295289,-4.96237823389833));
#109507=CARTESIAN_POINT('Ctrl Pts',(-16.9362777748711,18.0930122911458,
-4.96191159038382));
#109508=CARTESIAN_POINT('Ctrl Pts',(-16.9343972010295,18.0960419374689,
-4.9616956726169));
#109509=CARTESIAN_POINT('Ctrl Pts',(-16.9301550168041,18.1029148838485,
-4.96120546042073));
#109510=CARTESIAN_POINT('Ctrl Pts',(-16.927798042358,18.1067609699994,-4.96093086834725));
#109511=CARTESIAN_POINT('Ctrl Pts',(-16.921743663612,18.1167116884139,-4.96021979833486));
#109512=CARTESIAN_POINT('Ctrl Pts',(-16.9180648406238,18.1228274809193,
-4.95978215306416));
#109513=CARTESIAN_POINT('Ctrl Pts',(-16.8956530086545,18.1605157820108,
-4.95708197459196));
#109514=CARTESIAN_POINT('Ctrl Pts',(-16.8777141751826,18.1925505340961,
-4.95477313849696));
#109515=CARTESIAN_POINT('Ctrl Pts',(-16.7812829005166,18.3757742940944,
-4.94155914478204));
#109516=CARTESIAN_POINT('Ctrl Pts',(-16.7204309672991,18.5355380342309,
-4.93006551385103));
#109517=CARTESIAN_POINT('Ctrl Pts',(-16.6563716337719,18.7935463910746,
-4.91278849619484));
#109518=CARTESIAN_POINT('Ctrl Pts',(-16.6396560513731,18.8876815297255,
-4.90672131456489));
#109519=CARTESIAN_POINT('Ctrl Pts',(-16.6270441935145,19.0039146054185,
-4.89953963636454));
#109520=CARTESIAN_POINT('Ctrl Pts',(-16.6250580902273,19.025228083011,-4.89823496983708));
#109521=CARTESIAN_POINT('Ctrl Pts',(-16.6226955351678,19.0555533177765,
-4.89639541802049));
#109522=CARTESIAN_POINT('Ctrl Pts',(-16.622052933817,19.0645424709978,-4.89585221337528));
#109523=CARTESIAN_POINT('Ctrl Pts',(-16.6210439409712,19.0800485174159,
-4.89491871662535));
#109524=CARTESIAN_POINT('Ctrl Pts',(-16.6206502548811,19.0865634520563,
-4.89452757288727));
#109525=CARTESIAN_POINT('Ctrl Pts',(-16.6199544827135,19.0990351691825,
-4.8937808047889));
#109526=CARTESIAN_POINT('Ctrl Pts',(-16.6196474293291,19.1049916016644,
-4.89342502824345));
#109527=CARTESIAN_POINT('Ctrl Pts',(-16.6189150546905,19.1204708000555,
-4.89250269354047));
#109528=CARTESIAN_POINT('Ctrl Pts',(-16.6185288673296,19.1299953503005,
-4.89193736605631));
#109529=CARTESIAN_POINT('Ctrl Pts',(-16.6174336269316,19.162415280981,-4.89002031478329));
#109530=CARTESIAN_POINT('Ctrl Pts',(-16.6170318187375,19.1853199238369,
-4.88867819975365));
#109531=CARTESIAN_POINT('Ctrl Pts',(-16.6167705015412,19.3848364057372,
-4.87708360917363));
#109532=CARTESIAN_POINT('Ctrl Pts',(-16.6386380161249,19.5607779961173,
-4.86759334118126));
#109533=CARTESIAN_POINT('Ctrl Pts',(-16.7033214164755,19.8155383417283,
-4.85328915377275));
#109534=CARTESIAN_POINT('Ctrl Pts',(-16.7296216245108,19.8977219923509,
-4.84856684807259));
#109535=CARTESIAN_POINT('Ctrl Pts',(-16.7744878253125,20.0131324782004,
-4.84149568318189));
#109536=CARTESIAN_POINT('Ctrl Pts',(-16.7890513645391,20.0478266770472,
-4.83930994886156));
#109537=CARTESIAN_POINT('Ctrl Pts',(-16.8076413156073,20.0890024920954,
-4.8366219235295));
#109538=CARTESIAN_POINT('Ctrl Pts',(-16.8107890657166,20.0958761808335,
-4.83616999940829));
#109539=CARTESIAN_POINT('Ctrl Pts',(-16.8157341373979,20.1065236182853,
-4.83546476126004));
#109540=CARTESIAN_POINT('Ctrl Pts',(-16.8175059682376,20.1103092327208,
-4.83521299280402));
#109541=CARTESIAN_POINT('Ctrl Pts',(-16.8208093443362,20.117312979696,-4.83474524795382));
#109542=CARTESIAN_POINT('Ctrl Pts',(-16.8223378094702,20.120532501233,-4.83452946253968));
#109543=CARTESIAN_POINT('Ctrl Pts',(-16.8258074053121,20.1277933911589,
-4.83404107224157));
#109544=CARTESIAN_POINT('Ctrl Pts',(-16.827753237573,20.1318324388157,-4.83376817918748));
#109545=CARTESIAN_POINT('Ctrl Pts',(-16.8335217755547,20.1437098000355,
-4.83296218729391));
#109546=CARTESIAN_POINT('Ctrl Pts',(-16.8373800481002,20.1515305974386,
-4.83242695134667));
#109547=CARTESIAN_POINT('Ctrl Pts',(-16.8651905788954,20.2070360913482,
-4.82859720603469));
#109548=CARTESIAN_POINT('Ctrl Pts',(-16.8908879536521,20.2538199726222,
-4.82520557095097));
#109549=CARTESIAN_POINT('Ctrl Pts',(-16.9273703885928,20.3146702716838,
-4.82062016617669));
#109550=CARTESIAN_POINT('Ctrl Pts',(-16.9366060600847,20.329648122504,-4.81947691282786));
#109551=CARTESIAN_POINT('Ctrl Pts',(-16.9719974396182,20.3854737364625,
-4.81516492702491));
#109552=CARTESIAN_POINT('Ctrl Pts',(-16.9993672338391,20.4255330415147,
-4.81196743665102));
#109553=CARTESIAN_POINT('Ctrl Pts',(-17.0928606654789,20.5527582809314,
-4.80153807568917));
#109554=CARTESIAN_POINT('Ctrl Pts',(-17.1643724611866,20.6357548753799,
-4.79430527611817));
#109555=CARTESIAN_POINT('Ctrl Pts',(-17.2810732760338,20.7516911134269,
-4.78373162680585));
#109556=CARTESIAN_POINT('Ctrl Pts',(-17.3216673750704,20.7889868661811,
-4.78024239991532));
#109557=CARTESIAN_POINT('Ctrl Pts',(-17.3898211554562,20.8468633750935,
-4.77468470372269));
#109558=CARTESIAN_POINT('Ctrl Pts',(-17.4165057514967,20.8684302005164,
-4.77257779349461));
#109559=CARTESIAN_POINT('Ctrl Pts',(-17.452272882883,20.8959277198318,-4.76984121630616));
#109560=CARTESIAN_POINT('Ctrl Pts',(-17.4608922236801,20.902449798389,-4.76918820698987));
#109561=CARTESIAN_POINT('Ctrl Pts',(-17.4750937144903,20.9130257186884,
-4.76812270140971));
#109562=CARTESIAN_POINT('Ctrl Pts',(-17.480646319645,20.9171187345743,-4.76770867567016));
#109563=CARTESIAN_POINT('Ctrl Pts',(-17.4914348499393,20.9249902383723,
-4.76690915978977));
#109564=CARTESIAN_POINT('Ctrl Pts',(-17.4966682443373,20.928772050429,-4.76652354329821));
#109565=CARTESIAN_POINT('Ctrl Pts',(-17.5087941194647,20.9374504135402,
-4.76563512590242));
#109566=CARTESIAN_POINT('Ctrl Pts',(-17.5156988242927,20.9423297573094,
-4.76513299104892));
#109567=CARTESIAN_POINT('Ctrl Pts',(-17.5343516773014,20.9553443166718,
-4.76378639286306));
#109568=CARTESIAN_POINT('Ctrl Pts',(-17.5461533971386,20.9634022529772,
-4.76294487085612));
#109569=CARTESIAN_POINT('Ctrl Pts',(-17.6551779317309,21.0362341542191,
-4.75526378553406));
#109570=CARTESIAN_POINT('Ctrl Pts',(-17.7575304245802,21.0929801282206,
-4.74874083189837));
#109571=CARTESIAN_POINT('Ctrl Pts',(-18.0124244107475,21.207873484547,-4.73343466735366));
#109572=CARTESIAN_POINT('Ctrl Pts',(-18.1679920385624,21.2574110480607,
-4.72483454736412));
#109573=CARTESIAN_POINT('Ctrl Pts',(-18.3595787487887,21.2948796631286,
-4.71362552949456));
#109574=CARTESIAN_POINT('Ctrl Pts',(-18.3916191808121,21.3003828842905,
-4.71172955135087));
#109575=CARTESIAN_POINT('Ctrl Pts',(-18.4309329495605,21.3062068570694,
-4.70936322705093));
#109576=CARTESIAN_POINT('Ctrl Pts',(-18.4380996147278,21.3072309914524,
-4.70893024446441));
#109577=CARTESIAN_POINT('Ctrl Pts',(-18.4493425548703,21.3087788321044,
-4.70824826004283));
#109578=CARTESIAN_POINT('Ctrl Pts',(-18.4534154197205,21.3093274725701,
-4.70800064394495));
#109579=CARTESIAN_POINT('Ctrl Pts',(-18.4610311638127,21.310330791771,-4.70753654253321));
#109580=CARTESIAN_POINT('Ctrl Pts',(-18.4645736050249,21.3107883645363,
-4.70732022258151));
#109581=CARTESIAN_POINT('Ctrl Pts',(-18.472662440328,21.3118123834415,-4.70682527057329));
#109582=CARTESIAN_POINT('Ctrl Pts',(-18.4772095099472,21.3123730353803,
-4.70654631663277));
#109583=CARTESIAN_POINT('Ctrl Pts',(-18.4911910424031,21.3140508952117,
-4.70568643692749));
#109584=CARTESIAN_POINT('Ctrl Pts',(-18.5006310832383,21.3151193404124,
-4.70510287186301));
#109585=CARTESIAN_POINT('Ctrl Pts',(-18.585489176585,21.3241457018089,-4.6998321930468));
#109586=CARTESIAN_POINT('Ctrl Pts',(-18.6612692340638,21.3281083857921,
-4.69495035632745));
#109587=CARTESIAN_POINT('Ctrl Pts',(-18.9220127555302,21.3277278977201,
-4.67789742716739));
#109588=CARTESIAN_POINT('Ctrl Pts',(-19.1061435778507,21.3032272344487,
-4.66550056075186));
#109589=CARTESIAN_POINT('Ctrl Pts',(-19.3361783441231,21.2412480017666,
-4.65047356627224));
#109590=CARTESIAN_POINT('Ctrl Pts',(-19.3870671384211,21.2254552162038,
-4.64717203415066));
#109591=CARTESIAN_POINT('Ctrl Pts',(-19.4491381314976,21.2035922108457,
-4.64317041112002));
#109592=CARTESIAN_POINT('Ctrl Pts',(-19.4609293599016,21.1993208951696,
-4.64241136204275));
#109593=CARTESIAN_POINT('Ctrl Pts',(-19.479505556347,21.1924044208384,-4.64121713601289));
#109594=CARTESIAN_POINT('Ctrl Pts',(-19.4863158855397,21.1898286494515,
-4.64077965532218));
#109595=CARTESIAN_POINT('Ctrl Pts',(-19.4990580064809,21.1849340938054,
-4.63996172408139));
#109596=CARTESIAN_POINT('Ctrl Pts',(-19.5049928695549,21.1826235838602,
-4.63958100164126));
#109597=CARTESIAN_POINT('Ctrl Pts',(-19.5182501137179,21.1773933733746,
-4.63873105058719));
#109598=CARTESIAN_POINT('Ctrl Pts',(-19.5255668200928,21.1744594754203,
-4.63826230578819));
#109599=CARTESIAN_POINT('Ctrl Pts',(-19.5440621743795,21.1669229061899,
-4.63707817819079));
#109600=CARTESIAN_POINT('Ctrl Pts',(-19.5552181928735,21.1622651870272,
-4.63636466096839));
#109601=CARTESIAN_POINT('Ctrl Pts',(-19.6186396612221,21.1351459941704,
-4.63231157404071));
#109602=CARTESIAN_POINT('Ctrl Pts',(-19.6700255571715,21.1106794793352,
-4.62904111383941));
#109603=CARTESIAN_POINT('Ctrl Pts',(-19.7441246037395,21.0716606925732,
-4.62431035120919));
#109604=CARTESIAN_POINT('Ctrl Pts',(-19.7676425881203,21.0586993795897,
-4.62280643641715));
#109605=CARTESIAN_POINT('Ctrl Pts',(-19.8912830483217,20.9874585490753,
-4.61486906495003));
#109606=CARTESIAN_POINT('Ctrl Pts',(-19.986740954256,20.9214823632751,-4.60864416855414));
#109607=CARTESIAN_POINT('Ctrl Pts',(-20.1382144281337,20.7972776432238,
-4.59796527147532));
#109608=CARTESIAN_POINT('Ctrl Pts',(-20.197172748877,20.7430634541797,-4.59356345628013));
#109609=CARTESIAN_POINT('Ctrl Pts',(-20.2779936572084,20.6598163158203,
-4.58692644359765));
#109610=CARTESIAN_POINT('Ctrl Pts',(-20.3024069196683,20.6333517557169,
-4.58483230703258));
#109611=CARTESIAN_POINT('Ctrl Pts',(-20.3310516797729,20.6006656617167,
-4.58224585839903));
#109612=CARTESIAN_POINT('Ctrl Pts',(-20.3359416188343,20.5950259265279,
-4.58179958556928));
#109613=CARTESIAN_POINT('Ctrl Pts',(-20.3435094032093,20.5862039040975,
-4.58110128113724));
#109614=CARTESIAN_POINT('Ctrl Pts',(-20.3462079251059,20.5830393224708,
-4.58085074662194));
#109615=CARTESIAN_POINT('Ctrl Pts',(-20.3512028426161,20.5771466545727,
-4.58038410999141));
#109616=CARTESIAN_POINT('Ctrl Pts',(-20.3535016768327,20.574420710601,-4.58016819132513));
#109617=CARTESIAN_POINT('Ctrl Pts',(-20.3586930668443,20.5682331370054,
-4.57967796734314));
#109618=CARTESIAN_POINT('Ctrl Pts',(-20.3615814373997,20.5647680796201,
-4.57940336432214));
#109619=CARTESIAN_POINT('Ctrl Pts',(-20.3701034393598,20.5544778957299,
-4.57858771918393));
#109620=CARTESIAN_POINT('Ctrl Pts',(-20.3757052908646,20.5476267438118,
-4.57804446437036));
#109621=CARTESIAN_POINT('Ctrl Pts',(-20.416896854037,20.4965992241032,-4.57399809228173));
#109622=CARTESIAN_POINT('Ctrl Pts',(-20.4507378826997,20.4510471804908,
-4.57038527969595));
#109623=CARTESIAN_POINT('Ctrl Pts',(-20.517595504503,20.3530630292599,-4.56270258985737));
#109624=CARTESIAN_POINT('Ctrl Pts',(-20.5502243660562,20.3004261541394,
-4.55862492025321));
#109625=CARTESIAN_POINT('Ctrl Pts',(-20.6341053630717,20.1508409512255,
-4.5472967590275));
#109626=CARTESIAN_POINT('Ctrl Pts',(-20.6802112915795,20.0512181100901,
-4.54004817867238));
#109627=CARTESIAN_POINT('Ctrl Pts',(-20.7376833194159,19.8965708333749,
-4.52944135634561));
#109628=CARTESIAN_POINT('Ctrl Pts',(-20.7549277192372,19.8439345920452,
-4.52593485085462));
#109629=CARTESIAN_POINT('Ctrl Pts',(-20.7795153163776,19.7575720471792,
-4.52035286679903));
#109630=CARTESIAN_POINT('Ctrl Pts',(-20.7881324556578,19.7242387217262,
-4.5182385271321));
#109631=CARTESIAN_POINT('Ctrl Pts',(-20.7983855413429,19.680167832704,-4.51549385997609));
#109632=CARTESIAN_POINT('Ctrl Pts',(-20.8007569904306,19.6696084036162,
-4.51484001718692));
#109633=CARTESIAN_POINT('Ctrl Pts',(-20.8045078944324,19.6522863958362,
-4.51377350019948));
#109634=CARTESIAN_POINT('Ctrl Pts',(-20.8059354156874,19.6455345314609,
-4.51335929091796));
#109635=CARTESIAN_POINT('Ctrl Pts',(-20.8086343583903,19.6324533815842,
-4.512559661088));
#109636=CARTESIAN_POINT('Ctrl Pts',(-20.8099098928683,19.6261250317416,
-4.51217411292849));
#109637=CARTESIAN_POINT('Ctrl Pts',(-20.812787627958,19.6115026265349,-4.51128619626175));
#109638=CARTESIAN_POINT('Ctrl Pts',(-20.8143691798414,19.6032045827547,
-4.510784491395));
#109639=CARTESIAN_POINT('Ctrl Pts',(-20.818487729919,19.5808694012497,-4.50943980732034));
#109640=CARTESIAN_POINT('Ctrl Pts',(-20.8209326214634,19.5668155680512,
-4.50859975621447));
#109641=CARTESIAN_POINT('Ctrl Pts',(-20.8418093123264,19.4391846314612,
-4.50102309292269));
#109642=CARTESIAN_POINT('Ctrl Pts',(-20.8510962907031,19.3242992172063,
-4.49459289099642));
#109643=CARTESIAN_POINT('Ctrl Pts',(-20.8508421937423,19.0229639402604,
-4.47808646799875));
#109644=CARTESIAN_POINT('Ctrl Pts',(-20.8261075478324,18.8375810118745,
-4.46831888325726));
#109645=CARTESIAN_POINT('Ctrl Pts',(-20.7737437540966,18.6441344243448,
-4.45654192610075));
#109646=CARTESIAN_POINT('Ctrl Pts',(-20.7698906310994,18.6304481272354,
-4.45569953652088));
#109647=CARTESIAN_POINT('Ctrl Pts',(-20.7643392702254,18.6114648718975,
-4.45451699730324));
#109648=CARTESIAN_POINT('Ctrl Pts',(-20.7627574776398,18.6061338847515,
-4.45418335222364));
#109649=CARTESIAN_POINT('Ctrl Pts',(-20.7601843571559,18.5975855522441,
-4.45364575121933));
#109650=CARTESIAN_POINT('Ctrl Pts',(-20.7592063131376,18.5943641895252,
-4.45344256784534));
#109651=CARTESIAN_POINT('Ctrl Pts',(-20.7571469223496,18.5876389673479,
-4.4530171162032));
#109652=CARTESIAN_POINT('Ctrl Pts',(-20.7560641552701,18.5841355826974,
-4.45279476244682));
#109653=CARTESIAN_POINT('Ctrl Pts',(-20.7534222720431,18.5756656114123,
-4.45225546737612));
#109654=CARTESIAN_POINT('Ctrl Pts',(-20.7518539336428,18.5707019449483,
-4.45193798991217));
#109655=CARTESIAN_POINT('Ctrl Pts',(-20.7463005682226,18.5533490303559,
-4.45082319401964));
#109656=CARTESIAN_POINT('Ctrl Pts',(-20.7422197096073,18.5409910796789,
-4.45002052948399));
#109657=CARTESIAN_POINT('Ctrl Pts',(-20.7330366708962,18.5140201227554,
-4.44825071070825));
#109658=CARTESIAN_POINT('Ctrl Pts',(-20.7278880991585,18.4994251989497,
-4.44728132108652));
#109659=CARTESIAN_POINT('Ctrl Pts',(-20.722580615654,18.4848897225317,-4.44630506752222));
#109660=CARTESIAN_POINT('Origin',(-18.734,19.211,0.));
#109661=CARTESIAN_POINT('',(-20.7225806137986,18.4848897174502,-3.64442447432525));
#109662=CARTESIAN_POINT('',(-20.7225805460717,18.4848895319684,-3.86819362763421));
#109663=CARTESIAN_POINT('',(-20.7225806137986,18.4848897174502,0.));
#109664=CARTESIAN_POINT('',(-20.8509990913949,19.212945854356,-3.91098517251486));
#109665=CARTESIAN_POINT('Ctrl Pts',(-20.7225805460717,18.4848895319684,
-3.86819362763421));
#109666=CARTESIAN_POINT('Ctrl Pts',(-20.7339918661314,18.5161414283049,
-3.87027305953112));
#109667=CARTESIAN_POINT('Ctrl Pts',(-20.7446701890291,18.5476725148875,
-3.87233005867685));
#109668=CARTESIAN_POINT('Ctrl Pts',(-20.7593062383098,18.5945001734164,
-3.87532606019889));
#109669=CARTESIAN_POINT('Ctrl Pts',(-20.7638398855016,18.6095954311567,
-3.87628298084949));
#109670=CARTESIAN_POINT('Ctrl Pts',(-20.7704399629066,18.6324963854922,
-3.87772165193606));
#109671=CARTESIAN_POINT('Ctrl Pts',(-20.7726309379284,18.6402653363781,
-3.87820745032604));
#109672=CARTESIAN_POINT('Ctrl Pts',(-20.7764755276552,18.6542024643816,
-3.87907496958561));
#109673=CARTESIAN_POINT('Ctrl Pts',(-20.7781457595611,18.6603659184232,
-3.87945722668699));
#109674=CARTESIAN_POINT('Ctrl Pts',(-20.7816286851116,18.6734528061553,
-3.88026597292423));
#109675=CARTESIAN_POINT('Ctrl Pts',(-20.78343421329,18.6803780771307,-3.88069222567083));
#109676=CARTESIAN_POINT('Ctrl Pts',(-20.7870375877586,18.6944919473566,
-3.88155750779302));
#109677=CARTESIAN_POINT('Ctrl Pts',(-20.7888328801823,18.7016811000631,
-3.88199644993303));
#109678=CARTESIAN_POINT('Ctrl Pts',(-20.7932123060644,18.7196184020906,
-3.88308722853753));
#109679=CARTESIAN_POINT('Ctrl Pts',(-20.7957500889239,18.7303777222018,
-3.88373758024108));
#109680=CARTESIAN_POINT('Ctrl Pts',(-20.8334344277575,18.8959395700739,
-3.89368678770169));
#109681=CARTESIAN_POINT('Ctrl Pts',(-20.8511450350875,19.0541908602725,
-3.90236293223036));
#109682=CARTESIAN_POINT('Ctrl Pts',(-20.8509991056219,19.2129459691744,
-3.9109852020952));
#109683=CARTESIAN_POINT('Ctrl Pts',(-20.8509991057286,19.2129458531049,
-3.91098519579126));
#109684=CARTESIAN_POINT('Ctrl Pts',(-20.850867753823,19.355850713657,-3.91874661073577));
#109685=CARTESIAN_POINT('Ctrl Pts',(-20.8362669050489,19.4983604443446,
-3.92644252221242));
#109686=CARTESIAN_POINT('Ctrl Pts',(-20.8054595308778,19.6478519609443,
-3.93541366789966));
#109687=CARTESIAN_POINT('Ctrl Pts',(-20.8034239064502,19.6573954653553,
-3.93599045272699));
#109688=CARTESIAN_POINT('Ctrl Pts',(-20.8001171080786,19.6723896595962,
-3.93690356019448));
#109689=CARTESIAN_POINT('Ctrl Pts',(-20.7988901457165,19.6778500903219,
-3.93723753031756));
#109690=CARTESIAN_POINT('Ctrl Pts',(-20.796524907932,19.688184508945,-3.9378724508969));
#109691=CARTESIAN_POINT('Ctrl Pts',(-20.7953909685151,19.6930594622758,
-3.93817315943133));
#109692=CARTESIAN_POINT('Ctrl Pts',(-20.7934047157095,19.7014634516889,
-3.9386937048062));
#109693=CARTESIAN_POINT('Ctrl Pts',(-20.7925605836276,19.7049944371324,
-3.93891307202772));
#109694=CARTESIAN_POINT('Ctrl Pts',(-20.7909043902426,19.7118442907665,
-3.93933993107386));
#109695=CARTESIAN_POINT('Ctrl Pts',(-20.790093375697,19.7151633705692,-3.9395473563947));
#109696=CARTESIAN_POINT('Ctrl Pts',(-20.7878794157588,19.7241298146693,
-3.94010928592489));
#109697=CARTESIAN_POINT('Ctrl Pts',(-20.7864612271095,19.7297733325405,
-3.94046465583406));
#109698=CARTESIAN_POINT('Ctrl Pts',(-20.7810862687942,19.7507952962876,
-3.94179451832977));
#109699=CARTESIAN_POINT('Ctrl Pts',(-20.7769798907992,19.7661344748211,
-3.94277711452664));
#109700=CARTESIAN_POINT('Ctrl Pts',(-20.7391454582484,19.9013547930535,
-3.9515386807508));
#109701=CARTESIAN_POINT('Ctrl Pts',(-20.6950755517545,20.0180780298046,
-3.95978243884308));
#109702=CARTESIAN_POINT('Ctrl Pts',(-20.610136300618,20.1942889213471,-3.9727087389708));
#109703=CARTESIAN_POINT('Ctrl Pts',(-20.576054047705,20.256744816396,-3.97739737811818));
#109704=CARTESIAN_POINT('Ctrl Pts',(-20.4899911222872,20.3971448593993,
-3.98809703190452));
#109705=CARTESIAN_POINT('Ctrl Pts',(-20.4358500575675,20.4735984462119,
-3.99404315000294));
#109706=CARTESIAN_POINT('Ctrl Pts',(-20.3628825375995,20.5633753163385,
-4.00115615185354));
#109707=CARTESIAN_POINT('Ctrl Pts',(-20.3486769825774,20.580304793528,-4.00250405331161));
#109708=CARTESIAN_POINT('Ctrl Pts',(-20.3295476156363,20.6023904871968,
-4.00427189747669));
#109709=CARTESIAN_POINT('Ctrl Pts',(-20.3248595492177,20.6077482157587,
-4.00470150638706));
#109710=CARTESIAN_POINT('Ctrl Pts',(-20.3155382914039,20.6182931476713,
-4.00554858295229));
#109711=CARTESIAN_POINT('Ctrl Pts',(-20.3109063895642,20.6234813666053,
-4.00596609667235));
#109712=CARTESIAN_POINT('Ctrl Pts',(-20.3019392991922,20.63342636798,-4.00676788458745));
#109713=CARTESIAN_POINT('Ctrl Pts',(-20.2976078285496,20.6381863852303,
-4.00715230863392));
#109714=CARTESIAN_POINT('Ctrl Pts',(-20.287625817159,20.649056005087,-4.00803171756957));
#109715=CARTESIAN_POINT('Ctrl Pts',(-20.2819607997217,20.6551522146411,
-4.00852607981863));
#109716=CARTESIAN_POINT('Ctrl Pts',(-20.2667829295621,20.6712934226505,
-4.00983822117618));
#109717=CARTESIAN_POINT('Ctrl Pts',(-20.257207211776,20.6812789507222,-4.01065329248753));
#109718=CARTESIAN_POINT('Ctrl Pts',(-20.1814300812609,20.7587641498101,
-4.01700635350522));
#109719=CARTESIAN_POINT('Ctrl Pts',(-20.1108679839604,20.8218586141094,
-4.02234301004089));
#109720=CARTESIAN_POINT('Ctrl Pts',(-19.95614958634,20.9425827669569,-4.03318418439675));
#109721=CARTESIAN_POINT('Ctrl Pts',(-19.8715808680843,20.9992781203805,
-4.03865651750859));
#109722=CARTESIAN_POINT('Ctrl Pts',(-19.7137013728215,21.0893740505019,
-4.0485661575746));
#109723=CARTESIAN_POINT('Ctrl Pts',(-19.6419468757021,21.1250883784408,
-4.05297087424225));
#109724=CARTESIAN_POINT('Ctrl Pts',(-19.5352918338546,21.1708250111655,
-4.05960902222522));
#109725=CARTESIAN_POINT('Ctrl Pts',(-19.5018816381541,21.1841548647885,
-4.0617011052978));
#109726=CARTESIAN_POINT('Ctrl Pts',(-19.4611837250776,21.1992022030791,
-4.06428317001842));
#109727=CARTESIAN_POINT('Ctrl Pts',(-19.4542035952326,21.2017413061604,
-4.06472720069057));
#109728=CARTESIAN_POINT('Ctrl Pts',(-19.4432708698648,21.2056531878449,
-4.06542472214234));
#109729=CARTESIAN_POINT('Ctrl Pts',(-19.4393272427994,21.2070510981656,
-4.06567674625059));
#109730=CARTESIAN_POINT('Ctrl Pts',(-19.4320171661059,21.2096179563189,
-4.0661447231962));
#109731=CARTESIAN_POINT('Ctrl Pts',(-19.4286518992927,21.2107900984174,
-4.06636048350092));
#109732=CARTESIAN_POINT('Ctrl Pts',(-19.4210513783714,21.2134159043103,
-4.06684850522044));
#109733=CARTESIAN_POINT('Ctrl Pts',(-19.4168144870604,21.2148646226142,
-4.06712105287655));
#109734=CARTESIAN_POINT('Ctrl Pts',(-19.4043369949964,21.2190868789935,
-4.06792510144432));
#109735=CARTESIAN_POINT('Ctrl Pts',(-19.3960839826243,21.221823063935,-4.06845872440251));
#109736=CARTESIAN_POINT('Ctrl Pts',(-19.3375454000889,21.2408313666465,
-4.07225524890462));
#109737=CARTESIAN_POINT('Ctrl Pts',(-19.2866869885862,21.2552647843692,
-4.07561344863672));
#109738=CARTESIAN_POINT('Ctrl Pts',(-19.2204507581921,21.2714100897796,
-4.08001813576164));
#109739=CARTESIAN_POINT('Ctrl Pts',(-19.2055158934127,21.2748790720485,
-4.08101333744537));
#109740=CARTESIAN_POINT('Ctrl Pts',(-19.0333978799346,21.3128919203837,
-4.09249706823895));
#109741=CARTESIAN_POINT('Ctrl Pts',(-18.8727842150772,21.3295693034362,
-4.10329751587653));
#109742=CARTESIAN_POINT('Ctrl Pts',(-18.6568162402587,21.3273078474708,
-4.11717923825511));
#109743=CARTESIAN_POINT('Ctrl Pts',(-18.6018389500776,21.3245871197092,
-4.12066313369305));
#109744=CARTESIAN_POINT('Ctrl Pts',(-18.5130216741427,21.3167119886622,
-4.12620530749371));
#109745=CARTESIAN_POINT('Ctrl Pts',(-18.4790935954973,21.312874719827,-4.12830208991675));
#109746=CARTESIAN_POINT('Ctrl Pts',(-18.4348180102212,21.306779207003,-4.13101329655986));
#109747=CARTESIAN_POINT('Ctrl Pts',(-18.4243752397669,21.3052618894685,
-4.13165093414245));
#109748=CARTESIAN_POINT('Ctrl Pts',(-18.4070455278146,21.3026114545042,
-4.13270616650376));
#109749=CARTESIAN_POINT('Ctrl Pts',(-18.4001521513913,21.3015222599364,
-4.13312514446392));
#109750=CARTESIAN_POINT('Ctrl Pts',(-18.3869200970723,21.2993643981073,
-4.13392794825625));
#109751=CARTESIAN_POINT('Ctrl Pts',(-18.3805806637557,21.2983009108593,
-4.13431193354371));
#109752=CARTESIAN_POINT('Ctrl Pts',(-18.366096296104,21.2958031704144,-4.13518785563192));
#109753=CARTESIAN_POINT('Ctrl Pts',(-18.3579546928115,21.2943500245073,
-4.13567918663906));
#109754=CARTESIAN_POINT('Ctrl Pts',(-18.3363902971673,21.2903705948904,
-4.13697797063632));
#109755=CARTESIAN_POINT('Ctrl Pts',(-18.3229829435348,21.2877620323529,
-4.13778280380238));
#109756=CARTESIAN_POINT('Ctrl Pts',(-18.2236278534332,21.2674314331196,
-4.14372894601878));
#109757=CARTESIAN_POINT('Ctrl Pts',(-18.1388255651056,21.2445092882201,
-4.14869838640902));
#109758=CARTESIAN_POINT('Ctrl Pts',(-17.8817834971522,21.157565404442,-4.16373887211798));
#109759=CARTESIAN_POINT('Ctrl Pts',(-17.7162961194409,21.0763834248619,
-4.17333900079684));
#109760=CARTESIAN_POINT('Ctrl Pts',(-17.5291761549508,20.9521986035126,
-4.18611989109039));
#109761=CARTESIAN_POINT('Ctrl Pts',(-17.4956531643278,20.928518468108,-4.18849791955397));
#109762=CARTESIAN_POINT('Ctrl Pts',(-17.4566477509203,20.8992299114168,
-4.19139895718403));
#109763=CARTESIAN_POINT('Ctrl Pts',(-17.450479185991,20.8945448665962,-4.19186185463731));
#109764=CARTESIAN_POINT('Ctrl Pts',(-17.4409900393778,20.8872553653996,
-4.19258054501992));
#109765=CARTESIAN_POINT('Ctrl Pts',(-17.4376512266735,20.8846745996403,
-4.19283469628949));
#109766=CARTESIAN_POINT('Ctrl Pts',(-17.4315091613293,20.8798976292132,
-4.19330463565417));
#109767=CARTESIAN_POINT('Ctrl Pts',(-17.4287037245924,20.8777043272517,
-4.19352021839222));
#109768=CARTESIAN_POINT('Ctrl Pts',(-17.4224183459432,20.872764789715,-4.19400531532362));
#109769=CARTESIAN_POINT('Ctrl Pts',(-17.4189415126374,20.8700147153002,
-4.1942751002937));
#109770=CARTESIAN_POINT('Ctrl Pts',(-17.4100884139221,20.8629668543128,
-4.1949657047671));
#109771=CARTESIAN_POINT('Ctrl Pts',(-17.4047244717151,20.8586537689771,
-4.19538758426108));
#109772=CARTESIAN_POINT('Ctrl Pts',(-17.3738967156335,20.8336170022429,
-4.19783174972346));
#109773=CARTESIAN_POINT('Ctrl Pts',(-17.3488981942359,20.812330569676,-4.19989102638432));
#109774=CARTESIAN_POINT('Ctrl Pts',(-17.3101941905744,20.7777893528849,
-4.20319014382381));
#109775=CARTESIAN_POINT('Ctrl Pts',(-17.2961542531789,20.764914871017,-4.20441101973025));
#109776=CARTESIAN_POINT('Ctrl Pts',(-17.2642475181225,20.734854045894,-4.20723807508665));
#109777=CARTESIAN_POINT('Ctrl Pts',(-17.2465051133088,20.7175398786752,
-4.2088492569036));
#109778=CARTESIAN_POINT('Ctrl Pts',(-17.2259375552873,20.6967511623634,
-4.21076009609222));
#109779=CARTESIAN_POINT('Ctrl Pts',(-17.2228137848039,20.6935738013047,
-4.21105151378628));
#109780=CARTESIAN_POINT('Ctrl Pts',(-17.1169471842426,20.5852087646541,
-4.22096824518655));
#109781=CARTESIAN_POINT('Ctrl Pts',(-17.0254207144633,20.4695995216088,
-4.23080151624972));
#109782=CARTESIAN_POINT('Ctrl Pts',(-16.9048380449123,20.2796129005143,
-4.24528565078378));
#109783=CARTESIAN_POINT('Ctrl Pts',(-16.8667251726405,20.2115269131023,
-4.25019769506056));
#109784=CARTESIAN_POINT('Ctrl Pts',(-16.8240129462674,20.124239891412,-4.25615329087348));
#109785=CARTESIAN_POINT('Ctrl Pts',(-16.8158087092046,20.1068793751025,
-4.2573218374985));
#109786=CARTESIAN_POINT('Ctrl Pts',(-16.8042623546933,20.0815607554497,
-4.25900352774926));
#109787=CARTESIAN_POINT('Ctrl Pts',(-16.8007311027176,20.073690432823,-4.25952316859085));
#109788=CARTESIAN_POINT('Ctrl Pts',(-16.7946394142881,20.0598882472299,
-4.26042909863537));
#109789=CARTESIAN_POINT('Ctrl Pts',(-16.7920578627787,20.0539658799842,
-4.26081610780249));
#109790=CARTESIAN_POINT('Ctrl Pts',(-16.7871085860755,20.0424682854453,
-4.26156416036925));
#109791=CARTESIAN_POINT('Ctrl Pts',(-16.7847376009153,20.0368945380628,
-4.26192531206315));
#109792=CARTESIAN_POINT('Ctrl Pts',(-16.7791437389479,20.0235861238449,
-4.26278413862725));
#109793=CARTESIAN_POINT('Ctrl Pts',(-16.7759427818912,20.0158423098474,
-4.26328106659437));
#109794=CARTESIAN_POINT('Ctrl Pts',(-16.7646521127736,19.988061650068,-4.26505395761008));
#109795=CARTESIAN_POINT('Ctrl Pts',(-16.7568231245874,19.9679197863902,
-4.2663211393306));
#109796=CARTESIAN_POINT('Ctrl Pts',(-16.6831083100044,19.7693189137754,
-4.2786480987041));
#109797=CARTESIAN_POINT('Ctrl Pts',(-16.6412528391418,19.582875784331,-4.28879940722632));
#109798=CARTESIAN_POINT('Ctrl Pts',(-16.6232250431409,19.374344729596,-4.30022170439996));
#109799=CARTESIAN_POINT('Ctrl Pts',(-16.6218397323961,19.3553308972484,
-4.30126479176621));
#109800=CARTESIAN_POINT('Ctrl Pts',(-16.6169932428338,19.2735915825331,
-4.30576463364844));
#109801=CARTESIAN_POINT('Ctrl Pts',(-16.6160684380832,19.2107519804423,
-4.30926310047622));
#109802=CARTESIAN_POINT('Ctrl Pts',(-16.6188603926347,19.1170207153443,
-4.31465668960879));
#109803=CARTESIAN_POINT('Ctrl Pts',(-16.6204610476827,19.0860979029405,
-4.31646475486993));
#109804=CARTESIAN_POINT('Ctrl Pts',(-16.6232638245978,19.0481115448497,
-4.31873320122534));
#109805=CARTESIAN_POINT('Ctrl Pts',(-16.6238244702782,19.0410027016634,
-4.31915976938654));
#109806=CARTESIAN_POINT('Ctrl Pts',(-16.6247628177317,19.0298254916432,
-4.3198338709681));
#109807=CARTESIAN_POINT('Ctrl Pts',(-16.6251164062439,19.0257550786701,
-4.32008007105755));
#109808=CARTESIAN_POINT('Ctrl Pts',(-16.6258015267469,19.0181244375402,
-4.32054299049901));
#109809=CARTESIAN_POINT('Ctrl Pts',(-16.6261302959739,19.0145640170673,
-4.32075955342447));
#109810=CARTESIAN_POINT('Ctrl Pts',(-16.6269044006765,19.0064065832896,
-4.32125701920273));
#109811=CARTESIAN_POINT('Ctrl Pts',(-16.627355759526,19.0018101962475,-4.32153825659306));
#109812=CARTESIAN_POINT('Ctrl Pts',(-16.6288006813727,18.9875750174225,
-4.32241208012259));
#109813=CARTESIAN_POINT('Ctrl Pts',(-16.6298453679556,18.9779417020514,
-4.3230074286903));
#109814=CARTESIAN_POINT('Ctrl Pts',(-16.6419739042845,18.8728385405845,
-4.32954421755733));
#109815=CARTESIAN_POINT('Ctrl Pts',(-16.6594796819683,18.7782328137331,
-4.33579614055746));
#109816=CARTESIAN_POINT('Ctrl Pts',(-16.7131899272828,18.5687771107065,
-4.35003100339635));
#109817=CARTESIAN_POINT('Ctrl Pts',(-16.7528880351878,18.4551412718751,
-4.35802202617072));
#109818=CARTESIAN_POINT('Ctrl Pts',(-16.8275413648485,18.2885016939195,
-4.36982475130907));
#109819=CARTESIAN_POINT('Ctrl Pts',(-16.8555791961253,18.2326728059808,
-4.37379798928017));
#109820=CARTESIAN_POINT('Ctrl Pts',(-16.9043557041124,18.1454019907518,
-4.38002898448372));
#109821=CARTESIAN_POINT('Ctrl Pts',(-16.9235335981507,18.1131343172881,
-4.3823378146174));
#109822=CARTESIAN_POINT('Ctrl Pts',(-16.9495169516862,18.0719504519015,
-4.38529310840281));
#109823=CARTESIAN_POINT('Ctrl Pts',(-16.9555483241883,18.0625561541704,
-4.38596783290082));
#109824=CARTESIAN_POINT('Ctrl Pts',(-16.965469136165,18.0473693662882,-4.38705970168538));
#109825=CARTESIAN_POINT('Ctrl Pts',(-16.9693133374077,18.0415477125032,
-4.38747852396685));
#109826=CARTESIAN_POINT('Ctrl Pts',(-16.9767551984081,18.0303980197172,
-4.38828121813574));
#109827=CARTESIAN_POINT('Ctrl Pts',(-16.9803484827893,18.025067166252,-4.38866524846408));
#109828=CARTESIAN_POINT('Ctrl Pts',(-16.9886226992773,18.0129117051789,
-4.38954153362237));
#109829=CARTESIAN_POINT('Ctrl Pts',(-16.993319495717,18.006097983634,-4.39003318090292));
#109830=CARTESIAN_POINT('Ctrl Pts',(-17.0058841011221,17.9880971060124,
-4.39133335651856));
#109831=CARTESIAN_POINT('Ctrl Pts',(-17.0138206512216,17.9769582384652,
-4.39213925593046));
#109832=CARTESIAN_POINT('Ctrl Pts',(-17.0738934335507,17.8943524473931,
-4.39812779157076));
#109833=CARTESIAN_POINT('Ctrl Pts',(-17.1303586670236,17.8261347407728,
-4.40313560774494));
#109834=CARTESIAN_POINT('Ctrl Pts',(-17.2869184064686,17.6594523244136,
-4.41580640508079));
#109835=CARTESIAN_POINT('Ctrl Pts',(-17.3928134520657,17.5670528452157,
-4.42326352914345));
#109836=CARTESIAN_POINT('Ctrl Pts',(-17.5528127412453,17.453263537347,-4.43410166282991));
#109837=CARTESIAN_POINT('Ctrl Pts',(-17.599836630912,17.4225611885036,-4.43724511438607));
#109838=CARTESIAN_POINT('Ctrl Pts',(-17.6727199838165,17.379006112474,-4.44214098553462));
#109839=CARTESIAN_POINT('Ctrl Pts',(-17.6977155844563,17.3647521017972,
-4.44382414222081));
#109840=CARTESIAN_POINT('Ctrl Pts',(-17.7291130519032,17.3476858151744,
-4.44595321629649));
#109841=CARTESIAN_POINT('Ctrl Pts',(-17.7352499320191,17.3443892134516,
-4.44637005293538));
#109842=CARTESIAN_POINT('Ctrl Pts',(-17.7449795400622,17.3392243918855,
-4.4470321890741));
#109843=CARTESIAN_POINT('Ctrl Pts',(-17.7485616122287,17.3373360545226,
-4.44727623309904));
#109844=CARTESIAN_POINT('Ctrl Pts',(-17.7553228323461,17.3337965387391,
-4.44773742111767));
#109845=CARTESIAN_POINT('Ctrl Pts',(-17.7585007614253,17.3321431485381,
-4.44795442252671));
#109846=CARTESIAN_POINT('Ctrl Pts',(-17.765769891302,17.3283846313849,-4.44845130456129));
#109847=CARTESIAN_POINT('Ctrl Pts',(-17.7698637629372,17.3262847735014,
-4.44873151177234));
#109848=CARTESIAN_POINT('Ctrl Pts',(-17.7807378852902,17.3207518420043,
-4.44947671133752));
#109849=CARTESIAN_POINT('Ctrl Pts',(-17.7875297616807,17.3173419415997,
-4.44994309542689));
#109850=CARTESIAN_POINT('Ctrl Pts',(-17.8348595061783,17.293898005068,-4.45319887261588));
#109851=CARTESIAN_POINT('Ctrl Pts',(-17.8760087626475,17.2751322208204,
-4.45605849265602));
#109852=CARTESIAN_POINT('Ctrl Pts',(-17.9232435710595,17.2553929832994,
-4.45934827655616));
#109853=CARTESIAN_POINT('Ctrl Pts',(-17.9287732160307,17.2531096516789,
-4.45973351625342));
#109854=CARTESIAN_POINT('Ctrl Pts',(-18.080150210469,17.191351984878,-4.47028145726577));
#109855=CARTESIAN_POINT('Ctrl Pts',(-18.2321727060649,17.1483146819254,
-4.48087272568225));
#109856=CARTESIAN_POINT('Ctrl Pts',(-18.48917793289,17.1056829974042,-4.49778528429286));
#109857=CARTESIAN_POINT('Ctrl Pts',(-18.5918928706555,17.0962639513629,
-4.50430458954931));
#109858=CARTESIAN_POINT('Ctrl Pts',(-18.7097045144223,17.0940876277254,
-4.51149028355642));
#109859=CARTESIAN_POINT('Ctrl Pts',(-18.7245122508698,17.093969470554,-4.5123884112522));
#109860=CARTESIAN_POINT('Ctrl Pts',(-18.7470889492496,17.0940262090546,
-4.51375030993496));
#109861=CARTESIAN_POINT('Ctrl Pts',(-18.7548575018227,17.0940884951729,
-4.51421759231199));
#109862=CARTESIAN_POINT('Ctrl Pts',(-18.7689864260217,17.0942795609051,
-4.51506506775789));
#109863=CARTESIAN_POINT('Ctrl Pts',(-18.7753468677778,17.0943942489966,
-4.51544569748398));
#109864=CARTESIAN_POINT('Ctrl Pts',(-18.7890725173878,17.0947036360848,
-4.51626522605051));
#109865=CARTESIAN_POINT('Ctrl Pts',(-18.7964374378144,17.0949081185932,
-4.51670381355174));
#109866=CARTESIAN_POINT('Ctrl Pts',(-18.8163930954638,17.0955664496639,
-4.51788914297227));
#109867=CARTESIAN_POINT('Ctrl Pts',(-18.8289812177151,17.0960942558418,
-4.51863356399546));
#109868=CARTESIAN_POINT('Ctrl Pts',(-18.8900494265401,17.0992011247927,
-4.52222983657622));
#109869=CARTESIAN_POINT('Ctrl Pts',(-18.9384379720135,17.1033350455996,
-4.52503271372375));
#109870=CARTESIAN_POINT('Ctrl Pts',(-19.0271583474604,17.1139992203487,
-4.530111560573));
#109871=CARTESIAN_POINT('Ctrl Pts',(-19.0675242673698,17.1200394801967,
-4.53239924350846));
#109872=CARTESIAN_POINT('Ctrl Pts',(-19.2400317911566,17.1509762307576,
-4.5421260116405));
#109873=CARTESIAN_POINT('Ctrl Pts',(-19.3698055324556,17.1872616942401,
-4.54929584435369));
#109874=CARTESIAN_POINT('Ctrl Pts',(-19.5537915259837,17.2581647536107,
-4.56013215296928));
#109875=CARTESIAN_POINT('Ctrl Pts',(-19.6112868762622,17.2833096118014,
-4.5636256974789));
#109876=CARTESIAN_POINT('Ctrl Pts',(-19.6953392136571,17.324608536178,-4.56901242347579));
#109877=CARTESIAN_POINT('Ctrl Pts',(-19.7227978279106,17.3388556501038,
-4.57081880811596));
#109878=CARTESIAN_POINT('Ctrl Pts',(-19.7561871366722,17.357119400233,-4.5730853817558));
#109879=CARTESIAN_POINT('Ctrl Pts',(-19.7624240533147,17.360571999822,-4.57351182392422));
#109880=CARTESIAN_POINT('Ctrl Pts',(-19.7722074706896,17.3660525922125,
-4.57418577063532));
#109881=CARTESIAN_POINT('Ctrl Pts',(-19.7757658083966,17.3680594991958,
-4.57443194286774));
#109882=CARTESIAN_POINT('Ctrl Pts',(-19.7824276935411,17.3718422696254,
-4.5748948393983));
#109883=CARTESIAN_POINT('Ctrl Pts',(-19.7855325583813,17.3736157005773,
-4.57511140744684));
#109884=CARTESIAN_POINT('Ctrl Pts',(-19.7926381775716,17.3776981844922,
-4.5756089242432));
#109885=CARTESIAN_POINT('Ctrl Pts',(-19.7966358658039,17.3800124649442,
-4.57589020778408));
#109886=CARTESIAN_POINT('Ctrl Pts',(-19.8089993382034,17.3872238647522,
-4.57676431446321));
#109887=CARTESIAN_POINT('Ctrl Pts',(-19.8173389461491,17.3921652938784,
-4.57735990255948));
#109888=CARTESIAN_POINT('Ctrl Pts',(-19.907813927974,17.4466170017964,-4.58388414933513));
#109889=CARTESIAN_POINT('Ctrl Pts',(-19.9865190427039,17.5015912719082,
-4.59012195312501));
#109890=CARTESIAN_POINT('Ctrl Pts',(-20.1599368045378,17.6411434207766,
-4.60477496383618));
#109891=CARTESIAN_POINT('Ctrl Pts',(-20.2513330239269,17.7292947692964,
-4.61320501593265));
#109892=CARTESIAN_POINT('Ctrl Pts',(-20.3724508404403,17.8691489566997,
-4.62512679296181));
#109893=CARTESIAN_POINT('Ctrl Pts',(-20.4087701638008,17.9147626614726,
-4.62882514460463));
#109894=CARTESIAN_POINT('Ctrl Pts',(-20.4642424294529,17.9906614172447,
-4.6346755254161));
#109895=CARTESIAN_POINT('Ctrl Pts',(-20.4845889790407,18.0200324975842,
-4.63687123419375));
#109896=CARTESIAN_POINT('Ctrl Pts',(-20.5101992606089,18.0590774792216,
-4.63970428781388));
#109897=CARTESIAN_POINT('Ctrl Pts',(-20.5161437649286,18.0682957882801,
-4.64036708227154));
#109898=CARTESIAN_POINT('Ctrl Pts',(-20.5257284806865,18.0834158031858,
-4.6414444646975));
#109899=CARTESIAN_POINT('Ctrl Pts',(-20.5294117603708,18.089289840507,-4.64186064843995));
#109900=CARTESIAN_POINT('Ctrl Pts',(-20.5364622461458,18.1006575451075,
-4.64266154433391));
#109901=CARTESIAN_POINT('Ctrl Pts',(-20.5398333538535,18.1061486907982,
-4.64304639748499));
#109902=CARTESIAN_POINT('Ctrl Pts',(-20.5475262914819,18.1188088715705,
-4.64392911922893));
#109903=CARTESIAN_POINT('Ctrl Pts',(-20.5518307935931,18.1259883503612,
-4.64442634920298));
#109904=CARTESIAN_POINT('Ctrl Pts',(-20.5632211986325,18.1452444677378,
-4.64575116850041));
#109905=CARTESIAN_POINT('Ctrl Pts',(-20.5702301397846,18.1573663179927,
-4.6465759652113));
#109906=CARTESIAN_POINT('Ctrl Pts',(-20.6269889107861,18.2578165014144,
-4.65333768728098));
#109907=CARTESIAN_POINT('Ctrl Pts',(-20.6704588979085,18.3495497424042,
-4.6590410392201));
#109908=CARTESIAN_POINT('Ctrl Pts',(-20.7124627579728,18.4576170828737,
-4.66542622172685));
#109909=CARTESIAN_POINT('Ctrl Pts',(-20.7175926300245,18.4712292481404,
-4.66622485020144));
#109910=CARTESIAN_POINT('Ctrl Pts',(-20.7225805995351,18.4848896783871,
-4.66702134980151));
#109911=CARTESIAN_POINT('',(-20.8509999970067,19.2108919587094,-3.68920544123732));
#109912=CARTESIAN_POINT('Ctrl Pts',(-20.722580615654,18.4848897225317,-4.44630506752222));
#109913=CARTESIAN_POINT('Ctrl Pts',(-20.7059750647656,18.4394125028398,
-4.44325065798364));
#109914=CARTESIAN_POINT('Ctrl Pts',(-20.687813946497,18.3945171880631,-4.44012932677062));
#109915=CARTESIAN_POINT('Ctrl Pts',(-20.5919077352346,18.1790049071769,
-4.42474712639804));
#109916=CARTESIAN_POINT('Ctrl Pts',(-20.4932538286155,18.0185737177301,
-4.41214844665518));
#109917=CARTESIAN_POINT('Ctrl Pts',(-20.3393454720932,17.8298067791279,
-4.39674511146122));
#109918=CARTESIAN_POINT('Ctrl Pts',(-20.3022242257996,17.7877985027087,
-4.39326457188379));
#109919=CARTESIAN_POINT('Ctrl Pts',(-20.2551574930418,17.7386163329588,
-4.3891206613092));
#109920=CARTESIAN_POINT('Ctrl Pts',(-20.2467641308248,17.7299941001212,
-4.38839142612606));
#109921=CARTESIAN_POINT('Ctrl Pts',(-20.2327633239974,17.715854734914,-4.38719082706546));
#109922=CARTESIAN_POINT('Ctrl Pts',(-20.22719791156,17.7102965434215,-4.38671763388843));
#109923=CARTESIAN_POINT('Ctrl Pts',(-20.2170712326321,17.7002951106483,
-4.38586386176407));
#109924=CARTESIAN_POINT('Ctrl Pts',(-20.2125206719013,17.6958412070332,
-4.38548281432127));
#109925=CARTESIAN_POINT('Ctrl Pts',(-20.2027146322228,17.6863296991088,
-4.38466722087729));
#109926=CARTESIAN_POINT('Ctrl Pts',(-20.1974529597136,17.6812785763177,
-4.38423296041831));
#109927=CARTESIAN_POINT('Ctrl Pts',(-20.1830322479959,17.6675774231107,
-4.38305183146454));
#109928=CARTESIAN_POINT('Ctrl Pts',(-20.1738218416472,17.6589817071865,
-4.38230730786569));
#109929=CARTESIAN_POINT('Ctrl Pts',(-20.1246864970084,17.613939464373,-4.3783862137726));
#109930=CARTESIAN_POINT('Ctrl Pts',(-20.0834512253969,17.5789481009122,
-4.37527148823535));
#109931=CARTESIAN_POINT('Ctrl Pts',(-19.8904546629418,17.4274970951095,
-4.36137502640494));
#109932=CARTESIAN_POINT('Ctrl Pts',(-19.7246990486941,17.3303672047068,
-4.35135083627903));
#109933=CARTESIAN_POINT('Ctrl Pts',(-19.5328889714748,17.2504543797712,
-4.33979977051271));
#109934=CARTESIAN_POINT('Ctrl Pts',(-19.5175431875423,17.2442710479173,
-4.33887527946643));
#109935=CARTESIAN_POINT('Ctrl Pts',(-19.4525630585937,17.2189695945454,
-4.33495312214234));
#109936=CARTESIAN_POINT('Ctrl Pts',(-19.402293945906,17.2015472893796,-4.33190075803477));
#109937=CARTESIAN_POINT('Ctrl Pts',(-19.3430951221604,17.1834971006527,
-4.32822798148205));
#109938=CARTESIAN_POINT('Ctrl Pts',(-19.3347477731283,17.1810081325573,
-4.32770831536781));
#109939=CARTESIAN_POINT('Ctrl Pts',(-19.322083321175,17.1773168663385,-4.32691685596373));
#109940=CARTESIAN_POINT('Ctrl Pts',(-19.3177772525911,17.1760766109527,
-4.3266472213027));
#109941=CARTESIAN_POINT('Ctrl Pts',(-19.3100395890977,17.1738745515415,
-4.32616170707437));
#109942=CARTESIAN_POINT('Ctrl Pts',(-19.306609477271,17.1729077333922,-4.32594612289562));
#109943=CARTESIAN_POINT('Ctrl Pts',(-19.2991493967633,17.1708253398275,
-4.3254764697924));
#109944=CARTESIAN_POINT('Ctrl Pts',(-19.2951186120151,17.1697130561275,
-4.32522221903621));
#109945=CARTESIAN_POINT('Ctrl Pts',(-19.2837833131081,17.1666212230823,
-4.32450589440381));
#109946=CARTESIAN_POINT('Ctrl Pts',(-19.2764715266618,17.1646689139651,
-4.32404228847298));
#109947=CARTESIAN_POINT('Ctrl Pts',(-19.2326172483193,17.1532110035142,
-4.32125311852511));
#109948=CARTESIAN_POINT('Ctrl Pts',(-19.195838646655,17.1446458747669,-4.31887844929928));
#109949=CARTESIAN_POINT('Ctrl Pts',(-19.0738704374249,17.1196601704844,
-4.31093007550174));
#109950=CARTESIAN_POINT('Ctrl Pts',(-18.9879029346462,17.107492075934,-4.30521428398382));
#109951=CARTESIAN_POINT('Ctrl Pts',(-18.7261743169917,17.0867263830177,
-4.28786757581524));
#109952=CARTESIAN_POINT('Ctrl Pts',(-18.5498243946029,17.0947054605463,
-4.27632320851312));
#109953=CARTESIAN_POINT('Ctrl Pts',(-18.3538351297174,17.1282875791455,
-4.26408422115121));
#109954=CARTESIAN_POINT('Ctrl Pts',(-18.3312646901161,17.1325340532159,
-4.26268235718761));
#109955=CARTESIAN_POINT('Ctrl Pts',(-18.2994198446103,17.1390636754515,
-4.26071454750265));
#109956=CARTESIAN_POINT('Ctrl Pts',(-18.2900855430588,17.1410434777456,
-4.26013897797442));
#109957=CARTESIAN_POINT('Ctrl Pts',(-18.2749371557044,17.1443636270118,
-4.25920682258078));
#109958=CARTESIAN_POINT('Ctrl Pts',(-18.2691148663045,17.145665546026,-4.25884901077867));
#109959=CARTESIAN_POINT('Ctrl Pts',(-18.2569362435264,17.1484429097456,
-4.25810150661029));
#109960=CARTESIAN_POINT('Ctrl Pts',(-18.250581063225,17.1499231670467,-4.25771197316286));
#109961=CARTESIAN_POINT('Ctrl Pts',(-18.235473507884,17.1535157594482,-4.2567872037155));
#109962=CARTESIAN_POINT('Ctrl Pts',(-18.2267275190173,17.1556546038896,
-4.25625282683619));
#109963=CARTESIAN_POINT('Ctrl Pts',(-18.1972849081804,17.1630542184312,
-4.25445701876249));
#109964=CARTESIAN_POINT('Ctrl Pts',(-18.1766538907685,17.1685724302502,
-4.25320389844311));
#109965=CARTESIAN_POINT('Ctrl Pts',(-18.0646434242797,17.200355729808,-4.24642379584635));
#109966=CARTESIAN_POINT('Ctrl Pts',(-17.9750242182833,17.2324430964639,
-4.24109112091645));
#109967=CARTESIAN_POINT('Ctrl Pts',(-17.7316872667449,17.3385459389017,
-4.22648647745302));
#109968=CARTESIAN_POINT('Ctrl Pts',(-17.5843272499079,17.4252352698438,
-4.21752391412763));
#109969=CARTESIAN_POINT('Ctrl Pts',(-17.4194462256235,17.5511756457574,
-4.20567782967415));
#109970=CARTESIAN_POINT('Ctrl Pts',(-17.3905302472254,17.5744923895132,
-4.20352096207324));
#109971=CARTESIAN_POINT('Ctrl Pts',(-17.356788313006,17.603197684604,-4.20088735424399));
#109972=CARTESIAN_POINT('Ctrl Pts',(-17.351355787271,17.607867037987,-4.20045961333416));
#109973=CARTESIAN_POINT('Ctrl Pts',(-17.342535131102,17.6155267349443,-4.19975880212612));
#109974=CARTESIAN_POINT('Ctrl Pts',(-17.3391326419715,17.6185005577641,
-4.19948692657381));
#109975=CARTESIAN_POINT('Ctrl Pts',(-17.3330618671946,17.6238408812672,
-4.19899901699868));
#109976=CARTESIAN_POINT('Ctrl Pts',(-17.3303900175179,17.6262032505929,
-4.1987832911206));
#109977=CARTESIAN_POINT('Ctrl Pts',(-17.3246196760867,17.6313312526248,
-4.19831523404082));
#109978=CARTESIAN_POINT('Ctrl Pts',(-17.3215233919688,17.6340992168344,
-4.19806273133768));
#109979=CARTESIAN_POINT('Ctrl Pts',(-17.3129046318491,17.6418498225444,
-4.19735614318283));
#109980=CARTESIAN_POINT('Ctrl Pts',(-17.3074003041195,17.6468524274458,
-4.19690059048515));
#109981=CARTESIAN_POINT('Ctrl Pts',(-17.2757272576154,17.6759447152149,
-4.19425490305327));
#109982=CARTESIAN_POINT('Ctrl Pts',(-17.2501442479108,17.7006603428095,
-4.19202124248181));
#109983=CARTESIAN_POINT('Ctrl Pts',(-17.170173703602,17.7819130657839,-4.18475680991518));
#109984=CARTESIAN_POINT('Ctrl Pts',(-17.1183030536216,17.8408307157983,
-4.17960781614375));
#109985=CARTESIAN_POINT('Ctrl Pts',(-16.9535271245193,18.050393603072,-4.16201216346093));
#109986=CARTESIAN_POINT('Ctrl Pts',(-16.8574399055746,18.213181446054,-4.14960339835183));
#109987=CARTESIAN_POINT('Ctrl Pts',(-16.7756311802523,18.4066633888918,
-4.13668824432176));
#109988=CARTESIAN_POINT('Ctrl Pts',(-16.7674387063076,18.4269065410672,
-4.13535622741268));
#109989=CARTESIAN_POINT('Ctrl Pts',(-16.756524488722,18.4551227400292,-4.13352546182279));
#109990=CARTESIAN_POINT('Ctrl Pts',(-16.7535351252433,18.4629901652382,
-4.1330177513417));
#109991=CARTESIAN_POINT('Ctrl Pts',(-16.7484717503316,18.4765591416759,
-4.1321467723836));
#109992=CARTESIAN_POINT('Ctrl Pts',(-16.7463752024883,18.4822521217081,
-4.13178275285782));
#109993=CARTESIAN_POINT('Ctrl Pts',(-16.7420984657371,18.4940209588976,
-4.13103310100896));
#109994=CARTESIAN_POINT('Ctrl Pts',(-16.739921534041,18.5000979388113,-4.1306475805136));
#109995=CARTESIAN_POINT('Ctrl Pts',(-16.7349119396592,18.5142864679103,
-4.12975107784716));
#109996=CARTESIAN_POINT('Ctrl Pts',(-16.7321007820105,18.5224055307174,
-4.12924081421579));
#109997=CARTESIAN_POINT('Ctrl Pts',(-16.7232281509539,18.5485446979623,
-4.12760664635381));
#109998=CARTESIAN_POINT('Ctrl Pts',(-16.7173598591104,18.5666297390906,
-4.12648911944515));
#109999=CARTESIAN_POINT('Ctrl Pts',(-16.6890915632315,18.6579188087531,
-4.12091036382826));
#110000=CARTESIAN_POINT('Ctrl Pts',(-16.6704290036546,18.7322246281499,
-4.11657226150934));
#110001=CARTESIAN_POINT('Ctrl Pts',(-16.6348788992771,18.9152679743165,
-4.10620976643113));
#110002=CARTESIAN_POINT('Ctrl Pts',(-16.6223585149199,19.0246189832096,
-4.10029474841313));
#110003=CARTESIAN_POINT('Ctrl Pts',(-16.6158392212417,19.2047929696516,
-4.09047561005596));
#110004=CARTESIAN_POINT('Ctrl Pts',(-16.6168040098771,19.275215132183,-4.08661644390735));
#110005=CARTESIAN_POINT('Ctrl Pts',(-16.6243183281359,19.3932906483853,
-4.07993139949352));
#110006=CARTESIAN_POINT('Ctrl Pts',(-16.6289862469277,19.4410064665367,
-4.07717017350487));
#110007=CARTESIAN_POINT('Ctrl Pts',(-16.6362824266962,19.4961837374563,
-4.07386566470026));
#110008=CARTESIAN_POINT('Ctrl Pts',(-16.6373379659448,19.5038431188875,
-4.07340444064743));
#110009=CARTESIAN_POINT('Ctrl Pts',(-16.6390940231692,19.5160892927219,
-4.07266274657372));
#110010=CARTESIAN_POINT('Ctrl Pts',(-16.639767715947,19.5206799441147,-4.07238375076097));
#110011=CARTESIAN_POINT('Ctrl Pts',(-16.6409890215128,19.5288158470887,
-4.07188752889022));
#110012=CARTESIAN_POINT('Ctrl Pts',(-16.6415305602545,19.5323619646026,
-4.07167064878496));
#110013=CARTESIAN_POINT('Ctrl Pts',(-16.642699111912,19.5398857089864,-4.07120920979719));
#110014=CARTESIAN_POINT('Ctrl Pts',(-16.6433284510067,19.5438628662043,
-4.07096452691937));
#110015=CARTESIAN_POINT('Ctrl Pts',(-16.6450612823622,19.5546148278431,
-4.07030103345757));
#110016=CARTESIAN_POINT('Ctrl Pts',(-16.6461863728701,19.5613860318957,
-4.06988102750178));
#110017=CARTESIAN_POINT('Ctrl Pts',(-16.6519835356465,19.5952559195814,
-4.06776971895603));
#110018=CARTESIAN_POINT('Ctrl Pts',(-16.6571501298382,19.6222658739377,
-4.06605262054874));
#110019=CARTESIAN_POINT('Ctrl Pts',(-16.6736966018307,19.7004790971315,
-4.06099777990903));
#110020=CARTESIAN_POINT('Ctrl Pts',(-16.6864546820172,19.7513677512802,
-4.0576054311363));
#110021=CARTESIAN_POINT('Ctrl Pts',(-16.7401427624127,19.9361286281072,
-4.04502369798133));
#110022=CARTESIAN_POINT('Ctrl Pts',(-16.79243408485,20.0663388274407,-4.0356644091744));
#110023=CARTESIAN_POINT('Ctrl Pts',(-16.900499725592,20.2734155992247,-4.02055860764105));
#110024=CARTESIAN_POINT('Ctrl Pts',(-16.9492643995588,20.3534417420942,
-4.01465120724975));
#110025=CARTESIAN_POINT('Ctrl Pts',(-17.011125094351,20.4412771087141,-4.00809548250086));
#110026=CARTESIAN_POINT('Ctrl Pts',(-17.0191872008816,20.4524897433753,
-4.00725703246946));
#110027=CARTESIAN_POINT('Ctrl Pts',(-17.0322783287679,20.4703258062753,
-4.00592054850583));
#110028=CARTESIAN_POINT('Ctrl Pts',(-17.0372375582211,20.4769997440524,
-4.00541983201658));
#110029=CARTESIAN_POINT('Ctrl Pts',(-17.0461042224076,20.4887864641762,
-4.00453434448291));
#110030=CARTESIAN_POINT('Ctrl Pts',(-17.0499958671259,20.4939109423211,
-4.00414896296385));
#110031=CARTESIAN_POINT('Ctrl Pts',(-17.0581443281952,20.5045397882266,
-4.00334875529804));
#110032=CARTESIAN_POINT('Ctrl Pts',(-17.0624050450654,20.5100410789732,
-4.00293408937593));
#110033=CARTESIAN_POINT('Ctrl Pts',(-17.0735215436073,20.5242490626487,
-4.00186179521339));
#110034=CARTESIAN_POINT('Ctrl Pts',(-17.080418760196,20.5329231804923,-4.00120582230734));
#110035=CARTESIAN_POINT('Ctrl Pts',(-17.1104884222961,20.5701359542076,
-3.9983853637443));
#110036=CARTESIAN_POINT('Ctrl Pts',(-17.1343347539008,20.5981235437464,
-3.99624816700779));
#110037=CARTESIAN_POINT('Ctrl Pts',(-17.1994260566657,20.6706064196943,
-3.99065513274964));
#110038=CARTESIAN_POINT('Ctrl Pts',(-17.2418758012716,20.7139751442436,
-3.98724833320382));
#110039=CARTESIAN_POINT('Ctrl Pts',(-17.4049735342669,20.8668722265933,
-3.9748706233802));
#110040=CARTESIAN_POINT('Ctrl Pts',(-17.5362656309755,20.964182844412,-3.96628104198771));
#110041=CARTESIAN_POINT('Ctrl Pts',(-17.7270418601467,21.074063453883,-3.95393910670973));
#110042=CARTESIAN_POINT('Ctrl Pts',(-17.7778138397209,21.1006234864385,
-3.95066139504684));
#110043=CARTESIAN_POINT('Ctrl Pts',(-17.837614992549,21.128879453842,-3.94673759169723));
#110044=CARTESIAN_POINT('Ctrl Pts',(-17.8456586124068,21.1326183944585,
-3.94620852465209));
#110045=CARTESIAN_POINT('Ctrl Pts',(-17.8578318697443,21.1381841625579,
-3.94540553833769));
#110046=CARTESIAN_POINT('Ctrl Pts',(-17.8619443604361,21.1400485606969,
-3.94513387280138));
#110047=CARTESIAN_POINT('Ctrl Pts',(-17.8693154969831,21.1433618782294,
-3.94464618890131));
#110048=CARTESIAN_POINT('Ctrl Pts',(-17.8725718664981,21.144815732879,-3.94443047748826));
#110049=CARTESIAN_POINT('Ctrl Pts',(-17.8796309339621,21.1479459902976,
-3.94396227619773));
#110050=CARTESIAN_POINT('Ctrl Pts',(-17.883434847053,21.1496194031421,-3.94370961387164));
#110051=CARTESIAN_POINT('Ctrl Pts',(-17.89407163929,21.1542613951569,-3.94300213842293));
#110052=CARTESIAN_POINT('Ctrl Pts',(-17.9009152194604,21.1572050882865,
-3.94254585220056));
#110053=CARTESIAN_POINT('Ctrl Pts',(-17.9406995721641,21.1740696165025,
-3.93988749512523));
#110054=CARTESIAN_POINT('Ctrl Pts',(-17.9739712480407,21.1871892200748,
-3.93764141976049));
#110055=CARTESIAN_POINT('Ctrl Pts',(-18.0819002114488,21.2266188792609,
-3.93031837172091));
#110056=CARTESIAN_POINT('Ctrl Pts',(-18.1577034764265,21.2495863320778,
-3.92512120296864));
#110057=CARTESIAN_POINT('Ctrl Pts',(-18.4163930834376,21.3123823230059,
-3.90754875652674));
#110058=CARTESIAN_POINT('Ctrl Pts',(-18.6032674921169,21.3322305685399,
-3.89521656054633));
#110059=CARTESIAN_POINT('Ctrl Pts',(-18.8122853022599,21.3266659299767,
-3.88235981438239));
#110060=CARTESIAN_POINT('Ctrl Pts',(-18.8342203090713,21.3257403770736,
-3.88102059158552));
#110061=CARTESIAN_POINT('Ctrl Pts',(-18.8645581898705,21.3239871513727,
-3.87918159010935));
#110062=CARTESIAN_POINT('Ctrl Pts',(-18.8729758702505,21.3234502014291,
-3.87867274426296));
#110063=CARTESIAN_POINT('Ctrl Pts',(-18.887447045316,21.3224402355236,-3.87780033486632));
#110064=CARTESIAN_POINT('Ctrl Pts',(-18.8935020792573,21.3219914618044,
-3.87743601465167));
#110065=CARTESIAN_POINT('Ctrl Pts',(-18.9059877768061,21.3210120468745,
-3.87668621498173));
#110066=CARTESIAN_POINT('Ctrl Pts',(-18.9124181189947,21.3204780419723,
-3.87630084527842));
#110067=CARTESIAN_POINT('Ctrl Pts',(-18.9273880644794,21.3191659290448,
-3.87540549167693));
#110068=CARTESIAN_POINT('Ctrl Pts',(-18.9359256204032,21.3183653159795,
-3.87489622062075));
#110069=CARTESIAN_POINT('Ctrl Pts',(-18.9632838113231,21.3156320049038,
-3.87326848578385));
#110070=CARTESIAN_POINT('Ctrl Pts',(-18.9820838221897,21.3134988451238,
-3.87215632796617));
#110071=CARTESIAN_POINT('Ctrl Pts',(-19.076111084982,21.3015511723619,-3.86662268681255));
#110072=CARTESIAN_POINT('Ctrl Pts',(-19.1508051352289,21.2879495495841,
-3.86232201239333));
#110073=CARTESIAN_POINT('Ctrl Pts',(-19.3897571046286,21.2310227002554,
-3.84866507305576));
#110074=CARTESIAN_POINT('Ctrl Pts',(-19.5495534728259,21.17196273852,-3.83973272497251));
#110075=CARTESIAN_POINT('Ctrl Pts',(-19.7070546496591,21.0911347633064,
-3.82981948014393));
#110076=CARTESIAN_POINT('Ctrl Pts',(-19.7135192273012,21.0877749361364,
-3.82941042806757));
#110077=CARTESIAN_POINT('Ctrl Pts',(-19.7658461518226,21.0602351244969,
-3.82608076115078));
#110078=CARTESIAN_POINT('Ctrl Pts',(-19.8108195617706,21.0344132046163,
-3.82310258205018));
#110079=CARTESIAN_POINT('Ctrl Pts',(-19.862078072236,21.002424725352,-3.81951656572646));
#110080=CARTESIAN_POINT('Ctrl Pts',(-19.8693324423462,20.9978360090875,
-3.81900444039618));
#110081=CARTESIAN_POINT('Ctrl Pts',(-19.8802669595482,20.9908259639047,
-3.81822518775246));
#110082=CARTESIAN_POINT('Ctrl Pts',(-19.8839678855247,20.9884369934817,
-3.81796015980053));
#110083=CARTESIAN_POINT('Ctrl Pts',(-19.8905072638132,20.9841868118488,
-3.81748954560463));
#110084=CARTESIAN_POINT('Ctrl Pts',(-19.8933487235558,20.9823303074161,
-3.81728427480743));
#110085=CARTESIAN_POINT('Ctrl Pts',(-19.8962080372767,20.9804523104059,
-3.81707691835121));
#110086=CARTESIAN_POINT('Ctrl Pts',(-19.8962303296467,20.9804376681762,
-3.81707530166751));
#110087=CARTESIAN_POINT('Ctrl Pts',(-19.8962744428708,20.9804086922277,
-3.8170721023991));
#110088=CARTESIAN_POINT('Ctrl Pts',(-19.8962962637689,20.9803943585053,
-3.81707051981324));
#110089=CARTESIAN_POINT('Ctrl Pts',(-19.8963394627228,20.9803659808111,
-3.81706738666693));
#110090=CARTESIAN_POINT('Ctrl Pts',(-19.8963608410129,20.9803519367085,
-3.81706583609136));
#110091=CARTESIAN_POINT('Ctrl Pts',(-19.8964031821414,20.9803241203286,
-3.81706276498454));
#110092=CARTESIAN_POINT('Ctrl Pts',(-19.8964241447903,20.9803103481972,
-3.81706124446875));
#110093=CARTESIAN_POINT('Ctrl Pts',(-19.896465679522,20.9802830594733,-3.81705823168152));
#110094=CARTESIAN_POINT('Ctrl Pts',(-19.896486251433,20.9802695430135,-3.81705673942413));
#110095=CARTESIAN_POINT('Ctrl Pts',(-19.8965270271773,20.9802427509154,
-3.81705378152711));
#110096=CARTESIAN_POINT('Ctrl Pts',(-19.8965472311577,20.9802294751987,
-3.81705231587829));
#110097=CARTESIAN_POINT('Ctrl Pts',(-19.8965872927629,20.9802031503677,
-3.81704940962698));
#110098=CARTESIAN_POINT('Ctrl Pts',(-19.8966071503057,20.980190101324,-3.81704796903181));
#110099=CARTESIAN_POINT('Ctrl Pts',(-19.8966465386126,20.9801642170241,
-3.8170451114716));
#110100=CARTESIAN_POINT('Ctrl Pts',(-19.8966660694778,20.980151381717,-3.81704369450048));
#110101=CARTESIAN_POINT('Ctrl Pts',(-19.8967048233049,20.9801259125321,
-3.8170408828227));
#110102=CARTESIAN_POINT('Ctrl Pts',(-19.8967240461949,20.980113278716,-3.81703948812242));
#110103=CARTESIAN_POINT('Ctrl Pts',(-19.8967622007905,20.9800882015677,
-3.81703671977675));
#110104=CARTESIAN_POINT('Ctrl Pts',(-19.8967811327355,20.9800757580917,
-3.81703534611507));
#110105=CARTESIAN_POINT('Ctrl Pts',(-19.8968187226173,20.980051050374,-3.81703261860354));
#110106=CARTESIAN_POINT('Ctrl Pts',(-19.8968373802171,20.9800387863663,
-3.81703126477916));
#110107=CARTESIAN_POINT('Ctrl Pts',(-19.8968744356703,20.9800144282479,
-3.81702857591038));
#110108=CARTESIAN_POINT('Ctrl Pts',(-19.8968928337469,20.9800023340021,
-3.81702724085072));
#110109=CARTESIAN_POINT('Ctrl Pts',(-19.8969293855696,20.9799783053081,
-3.8170245883955));
#110110=CARTESIAN_POINT('Ctrl Pts',(-19.8969475389266,20.9799663711265,
-3.81702327102905));
#110111=CARTESIAN_POINT('Ctrl Pts',(-19.8969836133572,20.9799426546733,
-3.81702065308862));
#110112=CARTESIAN_POINT('Ctrl Pts',(-19.8970015349597,20.9799308720641,
-3.81701935247707));
#110113=CARTESIAN_POINT('Ctrl Pts',(-19.897037159241,20.9799074500023,-3.81701676707932));
#110114=CARTESIAN_POINT('Ctrl Pts',(-19.8970548619125,20.9798958105639,
-3.8170154822944));
#110115=CARTESIAN_POINT('Ctrl Pts',(-19.8970900604822,20.9798726668831,
-3.81701292767036));
#110116=CARTESIAN_POINT('Ctrl Pts',(-19.8971075562713,20.9798611627211,
-3.81701165783986));
#110117=CARTESIAN_POINT('Ctrl Pts',(-19.8971423522257,20.979838282288,-3.81700913231754));
#110118=CARTESIAN_POINT('Ctrl Pts',(-19.8971596524187,20.9798269060069,
-3.81700787662437));
#110119=CARTESIAN_POINT('Ctrl Pts',(-19.8971940678818,20.9798042743233,
-3.81700537860199));
#110120=CARTESIAN_POINT('Ctrl Pts',(-19.8972111832209,20.9797930188831,
-3.81700413626839));
#110121=CARTESIAN_POINT('Ctrl Pts',(-19.8972452388249,20.9797706224274,
-3.81700166425211));
#110122=CARTESIAN_POINT('Ctrl Pts',(-19.8972621792767,20.9797594812963,
-3.81700043455645));
#110123=CARTESIAN_POINT('Ctrl Pts',(-19.8972958956464,20.9797373065482,
-3.81699798705266));
#110124=CARTESIAN_POINT('Ctrl Pts',(-19.8973126712783,20.9797262731261,
-3.81699676926585));
#110125=CARTESIAN_POINT('Ctrl Pts',(-19.8973460657701,20.979704308711,-3.81699434501791));
#110126=CARTESIAN_POINT('Ctrl Pts',(-19.8973626851149,20.9796933774055,
-3.8169931385221));
#110127=CARTESIAN_POINT('Ctrl Pts',(-19.8973957775178,20.9796716103456,
-3.81699073609651));
#110128=CARTESIAN_POINT('Ctrl Pts',(-19.8974122498914,20.9796607750474,
-3.81698954021688));
#110129=CARTESIAN_POINT('Ctrl Pts',(-19.8974450561344,20.9796391949006,
-3.81698715846008));
#110130=CARTESIAN_POINT('Ctrl Pts',(-19.8974613898706,20.9796284501451,
-3.816985972593));
#110131=CARTESIAN_POINT('Ctrl Pts',(-19.8974939258221,20.9796070465062,
-3.81698361035562));
#110132=CARTESIAN_POINT('Ctrl Pts',(-19.8975101284448,20.9795963873599,
-3.81698243395613));
#110133=CARTESIAN_POINT('Ctrl Pts',(-19.9010366626355,20.9772763327961,
-3.81672638259861));
#110134=CARTESIAN_POINT('Ctrl Pts',(-19.90454007555,20.9749565149277,-3.81647080495603));
#110135=CARTESIAN_POINT('Ctrl Pts',(-19.9146438603917,20.9682228436645,
-3.81573028884217));
#110136=CARTESIAN_POINT('Ctrl Pts',(-19.9212262516046,20.9637823225676,
-3.81524360649331));
#110137=CARTESIAN_POINT('Ctrl Pts',(-19.9649805550544,20.9339058640675,
-3.81198090566468));
#110138=CARTESIAN_POINT('Ctrl Pts',(-20.0013547278463,20.9073281151426,
-3.80913489913387));
#110139=CARTESIAN_POINT('Ctrl Pts',(-20.1314017937029,20.805787560074,-3.79853955773096));
#110140=CARTESIAN_POINT('Ctrl Pts',(-20.2195034184797,20.7240621272268,
-3.79054128137616));
#110141=CARTESIAN_POINT('Ctrl Pts',(-20.3983278644827,20.5274235264769,
-3.77303710140993));
#110142=CARTESIAN_POINT('Ctrl Pts',(-20.4850526415925,20.4096607018668,
-3.76364162942936));
#110143=CARTESIAN_POINT('Ctrl Pts',(-20.5662145455078,20.2716045912233,
-3.75386354284211));
#110144=CARTESIAN_POINT('Ctrl Pts',(-20.573315395492,20.2592419239892,-3.75299760626831));
#110145=CARTESIAN_POINT('Ctrl Pts',(-20.5844228950989,20.2394432049183,
-3.75162590654722));
#110146=CARTESIAN_POINT('Ctrl Pts',(-20.5885107681369,20.2320534415698,
-3.75111723260238));
#110147=CARTESIAN_POINT('Ctrl Pts',(-20.5956451443323,20.2189722344933,
-3.75022253661821));
#110148=CARTESIAN_POINT('Ctrl Pts',(-20.5987100188426,20.2132909836896,
-3.74983586159837));
#110149=CARTESIAN_POINT('Ctrl Pts',(-20.6049980505754,20.2015064018072,
-3.74903766144175));
#110150=CARTESIAN_POINT('Ctrl Pts',(-20.6082174450039,20.1954011417382,
-3.74862627333748));
#110151=CARTESIAN_POINT('Ctrl Pts',(-20.6164099513422,20.1796789912534,
-3.74757228452061));
#110152=CARTESIAN_POINT('Ctrl Pts',(-20.6213392921878,20.1700394234663,
-3.74693123246866));
#110153=CARTESIAN_POINT('Ctrl Pts',(-20.6416483698221,20.1295609626519,
-3.74426040839557));
#110154=CARTESIAN_POINT('Ctrl Pts',(-20.656348412728,20.0983856682844,-3.74225439505245));
#110155=CARTESIAN_POINT('Ctrl Pts',(-20.6926986687246,20.0161479234924,
-3.73708223303656));
#110156=CARTESIAN_POINT('Ctrl Pts',(-20.7131157143972,19.9645683766573,
-3.73395603980857));
#110157=CARTESIAN_POINT('Ctrl Pts',(-20.7650951439492,19.8165055270243,
-3.72523304451047));
#110158=CARTESIAN_POINT('Ctrl Pts',(-20.7917797123911,19.7184721801879,
-3.71975545207146));
#110159=CARTESIAN_POINT('Ctrl Pts',(-20.8346708694905,19.5000398021504,
-3.70765144336622));
#110160=CARTESIAN_POINT('Ctrl Pts',(-20.8477626284588,19.3794088283171,
-3.70102956499715));
#110161=CARTESIAN_POINT('Ctrl Pts',(-20.8507280218477,19.2468325356147,
-3.69321457045652));
#110162=CARTESIAN_POINT('Ctrl Pts',(-20.8508915532428,19.2353233999873,
-3.69253165719203));
#110163=CARTESIAN_POINT('Ctrl Pts',(-20.8509827839472,19.2202512109919,
-3.69163079221853));
#110164=CARTESIAN_POINT('Ctrl Pts',(-20.8509953546732,19.2166886124106,
-3.69141737774716));
#110165=CARTESIAN_POINT('Ctrl Pts',(-20.8509997176845,19.2123441308279,
-3.69115652413364));
#110166=CARTESIAN_POINT('Ctrl Pts',(-20.8510000697334,19.2115622346711,
-3.69110955337614));
#110167=CARTESIAN_POINT('Ctrl Pts',(-20.850999988604,19.2107803400989,-3.6910625588116));
#110168=CARTESIAN_POINT('Ctrl Pts',(-20.8509999976816,19.2109009238279,
-3.6890562790225));
#110169=CARTESIAN_POINT('Ctrl Pts',(-20.8509997507685,19.2056250329455,
-3.68873698393553));
#110170=CARTESIAN_POINT('Ctrl Pts',(-20.8509797813958,19.2003491960952,
-3.68841768884856));
#110171=CARTESIAN_POINT('Ctrl Pts',(-20.8509400905189,19.1950735078034,
-3.68809839376159));
#110172=CARTESIAN_POINT('Ctrl Pts',(-20.8503947174663,19.1225828384675,
-3.68371111511857));
#110173=CARTESIAN_POINT('Ctrl Pts',(-20.8461205125477,19.0499787438565,
-3.67932383647555));
#110174=CARTESIAN_POINT('Ctrl Pts',(-20.8381029246807,18.9776764427882,
-3.67493655783253));
#110175=CARTESIAN_POINT('Ctrl Pts',(-20.8300957679091,18.9054682089396,
-3.67055498715589));
#110176=CARTESIAN_POINT('Ctrl Pts',(-20.8183549391171,18.8335614650894,
-3.66617341647925));
#110177=CARTESIAN_POINT('Ctrl Pts',(-20.8029178766155,18.7623711781205,
-3.66179184580261));
#110178=CARTESIAN_POINT('Ctrl Pts',(-20.7874985864815,18.6912628510425,
-3.6574153195368));
#110179=CARTESIAN_POINT('Ctrl Pts',(-20.7683916165293,18.6208698115597,
-3.65303879327099));
#110180=CARTESIAN_POINT('Ctrl Pts',(-20.745685938542,18.5515997538124,-3.64866226700518));
#110181=CARTESIAN_POINT('Ctrl Pts',(-20.7383572985718,18.5292416760561,
-3.64724966944521));
#110182=CARTESIAN_POINT('Ctrl Pts',(-20.7306541493028,18.5070005132541,
-3.64583707188523));
#110183=CARTESIAN_POINT('Ctrl Pts',(-20.7225806137986,18.4848897174502,
-3.64442447432525));
#110184=CARTESIAN_POINT('Origin',(-18.734,19.211,0.));
#110185=CARTESIAN_POINT('',(-20.7202231698227,18.4857291668959,-2.84456322999407));
#110186=CARTESIAN_POINT('',(-20.7225805974208,18.4848896725968,-3.06515445288237));
#110187=CARTESIAN_POINT('',(-20.7225806137986,18.4848897174502,0.));
#110188=CARTESIAN_POINT('Ctrl Pts',(-20.7225805974208,18.4848896725968,
-3.06515445288237));
#110189=CARTESIAN_POINT('Ctrl Pts',(-20.775012214741,18.6284828607934,-3.07512670877195));
#110190=CARTESIAN_POINT('Ctrl Pts',(-20.8117530652564,18.7773757226491,
-3.085373849156));
#110191=CARTESIAN_POINT('Ctrl Pts',(-20.8399080750925,18.9868384898001,
-3.09899376967294));
#110192=CARTESIAN_POINT('Ctrl Pts',(-20.8452891067731,19.0449985660853,
-3.10269880438067));
#110193=CARTESIAN_POINT('Ctrl Pts',(-20.8500786760388,19.1390322794493,
-3.10855849336733));
#110194=CARTESIAN_POINT('Ctrl Pts',(-20.8509926290692,19.1747954495418,
-3.11075700017239));
#110195=CARTESIAN_POINT('Ctrl Pts',(-20.8510022031441,19.221539806733,-3.11359308617401));
#110196=CARTESIAN_POINT('Ctrl Pts',(-20.8509191302513,19.2325132220007,
-3.11425618280915));
#110197=CARTESIAN_POINT('Ctrl Pts',(-20.8506443290578,19.250419142171,-3.11533393209238));
#110198=CARTESIAN_POINT('Ctrl Pts',(-20.8505038547006,19.2573521231421,
-3.11575018257836));
#110199=CARTESIAN_POINT('Ctrl Pts',(-20.8501671509656,19.2707252043125,
-3.11655112251225));
#110200=CARTESIAN_POINT('Ctrl Pts',(-20.849975581304,19.2771653353186,-3.11693595340708));
#110201=CARTESIAN_POINT('Ctrl Pts',(-20.8494626510919,19.2921125322765,
-3.11782712519268));
#110202=CARTESIAN_POINT('Ctrl Pts',(-20.8491193701468,19.3006187721233,
-3.11833277398264));
#110203=CARTESIAN_POINT('Ctrl Pts',(-20.847863432287,19.3276865154241,-3.11993717187166));
#110204=CARTESIAN_POINT('Ctrl Pts',(-20.8467576611286,19.3462384974586,
-3.12102987033051));
#110205=CARTESIAN_POINT('Ctrl Pts',(-20.843613922483,19.3894038934937,-3.12355755269016));
#110206=CARTESIAN_POINT('Ctrl Pts',(-20.8413892435542,19.4140012283545,
-3.12498673363693));
#110207=CARTESIAN_POINT('Ctrl Pts',(-20.8320826229699,19.5000814633134,
-3.12995533127274));
#110208=CARTESIAN_POINT('Ctrl Pts',(-20.8227356741548,19.561289781124,-3.13342816695607));
#110209=CARTESIAN_POINT('Ctrl Pts',(-20.7831185790056,19.7614667236369,
-3.14471626565864));
#110210=CARTESIAN_POINT('Ctrl Pts',(-20.7415412504979,19.8977869162543,
-3.15226972708296));
#110211=CARTESIAN_POINT('Ctrl Pts',(-20.6575318191133,20.0983454768993,
-3.16430899961774));
#110212=CARTESIAN_POINT('Ctrl Pts',(-20.6247655991321,20.1661751433871,
-3.16856365020628));
#110213=CARTESIAN_POINT('Ctrl Pts',(-20.5838856182396,20.2404183812028,
-3.1735867907708));
#110214=CARTESIAN_POINT('Ctrl Pts',(-20.5792539450497,20.2486978726146,
-3.17415229018995));
#110215=CARTESIAN_POINT('Ctrl Pts',(-20.5723045719363,20.2609267913955,
-3.17499588748264));
#110216=CARTESIAN_POINT('Ctrl Pts',(-20.5700293810929,20.2649004114961,
-3.17527131949992));
#110217=CARTESIAN_POINT('Ctrl Pts',(-20.5659565704835,20.2719603577674,
-3.17576308529832));
#110218=CARTESIAN_POINT('Ctrl Pts',(-20.5641640141925,20.2750495466917,
-3.17597909074816));
#110219=CARTESIAN_POINT('Ctrl Pts',(-20.5602911420992,20.2816850928805,
-3.17644486281203));
#110220=CARTESIAN_POINT('Ctrl Pts',(-20.5582083408837,20.2852298786632,
-3.17669478550824));
#110221=CARTESIAN_POINT('Ctrl Pts',(-20.5524255451225,20.295006486479,-3.17738707893546));
#110222=CARTESIAN_POINT('Ctrl Pts',(-20.5487038952051,20.301225341437,-3.17783082404308));
#110223=CARTESIAN_POINT('Ctrl Pts',(-20.5280542177102,20.3353321408251,
-3.18028263168886));
#110224=CARTESIAN_POINT('Ctrl Pts',(-20.5105162007989,20.3628433991225,
-3.18232723262178));
#110225=CARTESIAN_POINT('Ctrl Pts',(-20.40178357793,20.5250150383694,-3.19473512450942));
#110226=CARTESIAN_POINT('Ctrl Pts',(-20.295956055093,20.6492040214767,-3.20568691734734));
#110227=CARTESIAN_POINT('Ctrl Pts',(-20.0915016472688,20.8396550263871,
-3.22393800697634));
#110228=CARTESIAN_POINT('Ctrl Pts',(-19.9995963150936,20.9120589895192,
-3.23137712523197));
#110229=CARTESIAN_POINT('Ctrl Pts',(-19.8902556615087,20.9844052049271,
-3.23938257961643));
#110230=CARTESIAN_POINT('Ctrl Pts',(-19.8782592753593,20.9921692513918,
-3.24025053463299));
#110231=CARTESIAN_POINT('Ctrl Pts',(-19.8590411983013,21.0043328690579,
-3.24162481633562));
#110232=CARTESIAN_POINT('Ctrl Pts',(-19.8518703318491,21.0088115589598,
-3.24213407091119));
#110233=CARTESIAN_POINT('Ctrl Pts',(-19.8391760174011,21.0166346971543,
-3.24302944204619));
#110234=CARTESIAN_POINT('Ctrl Pts',(-19.8336637739074,21.0199970355959,
-3.24341621470033));
#110235=CARTESIAN_POINT('Ctrl Pts',(-19.8222308205539,21.0268992992335,
-3.24421428482523));
#110236=CARTESIAN_POINT('Ctrl Pts',(-19.8163080120847,21.030435613719,-3.24462544689818));
#110237=CARTESIAN_POINT('Ctrl Pts',(-19.801060512177,21.0394385946097,-3.24567816979294));
#110238=CARTESIAN_POINT('Ctrl Pts',(-19.7917109742872,21.0448629535321,
-3.24631818923801));
#110239=CARTESIAN_POINT('Ctrl Pts',(-19.7525150439798,21.067203937102,-3.24897895783253));
#110240=CARTESIAN_POINT('Ctrl Pts',(-19.7223002287249,21.0834659691048,
-3.25097617591453));
#110241=CARTESIAN_POINT('Ctrl Pts',(-19.6425552123937,21.1239175029515,
-3.2561205376204));
#110242=CARTESIAN_POINT('Ctrl Pts',(-19.5924513012576,21.1469204415304,
-3.25922828654674));
#110243=CARTESIAN_POINT('Ctrl Pts',(-19.4404219972875,21.209653104444,-3.26837302845841));
#110244=CARTESIAN_POINT('Ctrl Pts',(-19.3362575590134,21.2434696765374,
-3.27426129316222));
#110245=CARTESIAN_POINT('Ctrl Pts',(-19.1852135492876,21.2798674789338,
-3.28272017110981));
#110246=CARTESIAN_POINT('Ctrl Pts',(-19.1401414519775,21.2891855525484,
-3.28523620590521));
#110247=CARTESIAN_POINT('Ctrl Pts',(-19.073001551379,21.3007981888584,-3.28901509784947));
#110248=CARTESIAN_POINT('Ctrl Pts',(-19.0511428507339,21.3042269076325,
-3.29025024055008));
#110249=CARTESIAN_POINT('Ctrl Pts',(-18.978253818477,21.3144922634723,-3.29439637283993));
#110250=CARTESIAN_POINT('Ctrl Pts',(-18.9270320586601,21.3198094577491,
-3.29735453965841));
#110251=CARTESIAN_POINT('Ctrl Pts',(-18.8670520534064,21.3238324097688,
-3.30092250667448));
#110252=CARTESIAN_POINT('Ctrl Pts',(-18.8584286452259,21.3243577896704,
-3.3014379830703));
#110253=CARTESIAN_POINT('Ctrl Pts',(-18.845343308835,21.3250746465095,-3.3022243006764));
#110254=CARTESIAN_POINT('Ctrl Pts',(-18.8408834728445,21.3253048185702,
-3.30249302502683));
#110255=CARTESIAN_POINT('Ctrl Pts',(-18.8328642775101,21.3256932516972,
-3.30297757446185));
#110256=CARTESIAN_POINT('Ctrl Pts',(-18.8293052210298,21.3258566402184,
-3.30319310935092));
#110257=CARTESIAN_POINT('Ctrl Pts',(-18.8215562313466,21.3261927787466,
-3.30366344825236));
#110258=CARTESIAN_POINT('Ctrl Pts',(-18.8173662457479,21.3263620619827,
-3.30391843844027));
#110259=CARTESIAN_POINT('Ctrl Pts',(-18.8055579570647,21.3268040013217,
-3.30463889504533));
#110260=CARTESIAN_POINT('Ctrl Pts',(-18.7979387349794,21.3270479548772,
-3.30510592140441));
#110261=CARTESIAN_POINT('Ctrl Pts',(-18.7515937563836,21.3282813056429,
-3.30795910531823));
#110262=CARTESIAN_POINT('Ctrl Pts',(-18.7128507610393,21.328248672019,-3.3103969694704));
#110263=CARTESIAN_POINT('Ctrl Pts',(-18.5834923031677,21.3245890866357,
-3.31866562074778));
#110264=CARTESIAN_POINT('Ctrl Pts',(-18.4931149887585,21.3162039811179,
-3.32465026798381));
#110265=CARTESIAN_POINT('Ctrl Pts',(-18.3372625355312,21.2915752780926,
-3.33507719097317));
#110266=CARTESIAN_POINT('Ctrl Pts',(-18.2714988683308,21.2779512213385,
-3.33951171173244));
#110267=CARTESIAN_POINT('Ctrl Pts',(-18.0953552671279,21.232630759643,-3.35138293638831));
#110268=CARTESIAN_POINT('Ctrl Pts',(-17.9867140704593,21.1950436445113,
-3.35868689673394));
#110269=CARTESIAN_POINT('Ctrl Pts',(-17.8685880837743,21.1430855425856,
-3.36656625559629));
#110270=CARTESIAN_POINT('Ctrl Pts',(-17.8555936912105,21.1372125274513,
-3.3674323841291));
#110271=CARTESIAN_POINT('Ctrl Pts',(-17.8349986670949,21.1276525337581,
-3.36880432942311));
#110272=CARTESIAN_POINT('Ctrl Pts',(-17.8273592228718,21.1240506622157,
-3.3693130586054));
#110273=CARTESIAN_POINT('Ctrl Pts',(-17.813919174055,21.11761531111,-3.37020781879654));
#110274=CARTESIAN_POINT('Ctrl Pts',(-17.8081096296087,21.1148008546797,
-3.37059450308193));
#110275=CARTESIAN_POINT('Ctrl Pts',(-17.7961157028666,21.1089224634733,
-3.37139269076218));
#110276=CARTESIAN_POINT('Ctrl Pts',(-17.7899332414578,21.1058547673412,
-3.37180405728046));
#110277=CARTESIAN_POINT('Ctrl Pts',(-17.7740927566258,21.0978980525252,
-3.3728579252438));
#110278=CARTESIAN_POINT('Ctrl Pts',(-17.7644569541153,21.0929650542106,
-3.37349887872411));
#110279=CARTESIAN_POINT('Ctrl Pts',(-17.7243189894809,21.072026541128,-3.37616874133761));
#110280=CARTESIAN_POINT('Ctrl Pts',(-17.6941709200601,21.0553511632146,
-3.37817391360766));
#110281=CARTESIAN_POINT('Ctrl Pts',(-17.6166177366247,21.0099488348847,
-3.38334341493393));
#110282=CARTESIAN_POINT('Ctrl Pts',(-17.5699091969802,20.9800826125672,
-3.38646784241915));
#110283=CARTESIAN_POINT('Ctrl Pts',(-17.4344713874162,20.8857918156409,
-3.39564166942676));
#110284=CARTESIAN_POINT('Ctrl Pts',(-17.3495158114413,20.8162746262539,
-3.40154244090375));
#110285=CARTESIAN_POINT('Ctrl Pts',(-17.225310181684,20.6974138547889,-3.41090368402622));
#110286=CARTESIAN_POINT('Ctrl Pts',(-17.1822206234332,20.6523712729702,
-3.41431616019914));
#110287=CARTESIAN_POINT('Ctrl Pts',(-17.1041137128793,20.5631562324361,
-3.4209687322884));
#110288=CARTESIAN_POINT('Ctrl Pts',(-17.0687514768634,20.5193585000381,
-3.42419111435789));
#110289=CARTESIAN_POINT('Ctrl Pts',(-17.0299084709903,20.4671206474124,
-3.4280532717781));
#110290=CARTESIAN_POINT('Ctrl Pts',(-17.024682418431,20.4599997675315,-3.42858014025258));
#110291=CARTESIAN_POINT('Ctrl Pts',(-17.0168571005632,20.4491960990727,
-3.42938043207831));
#110292=CARTESIAN_POINT('Ctrl Pts',(-17.0142247101722,20.4455372689714,
-3.42965162410959));
#110293=CARTESIAN_POINT('Ctrl Pts',(-17.009530899628,20.4389690695605,-3.4301388000767));
#110294=CARTESIAN_POINT('Ctrl Pts',(-17.0074651277757,20.4360628753863,
-3.43035447975497));
#110295=CARTESIAN_POINT('Ctrl Pts',(-17.0030041564275,20.4297533420393,
-3.43082301017017));
#110296=CARTESIAN_POINT('Ctrl Pts',(-17.0006116797986,20.4263482010923,
-3.4310760355064));
#110297=CARTESIAN_POINT('Ctrl Pts',(-16.9939489536351,20.4168056473766,
-3.43178553014063));
#110298=CARTESIAN_POINT('Ctrl Pts',(-16.9897012045009,20.410652704489,-3.43224348589867));
#110299=CARTESIAN_POINT('Ctrl Pts',(-16.9650749828866,20.3745738607738,
-3.43493097030043));
#110300=CARTESIAN_POINT('Ctrl Pts',(-16.9454356177525,20.3441535347104,
-3.43720561419485));
#110301=CARTESIAN_POINT('Ctrl Pts',(-16.8845208226642,20.2442683094055,
-3.44466468408632));
#110302=CARTESIAN_POINT('Ctrl Pts',(-16.8464403662523,20.1729425754835,
-3.4499739400314));
#110303=CARTESIAN_POINT('Ctrl Pts',(-16.7350609161826,19.9321063296024,
-3.46749411760044));
#110304=CARTESIAN_POINT('Ctrl Pts',(-16.679811808078,19.7551413958542,-3.47965067302103));
#110305=CARTESIAN_POINT('Ctrl Pts',(-16.644420229391,19.5513505656333,-3.49237226884231));
#110306=CARTESIAN_POINT('Ctrl Pts',(-16.6409649746219,19.5294125731856,
-3.49372720568573));
#110307=CARTESIAN_POINT('Ctrl Pts',(-16.6366688351066,19.4990326387749,
-3.49558412386552));
#110308=CARTESIAN_POINT('Ctrl Pts',(-16.6355326196902,19.490634535199,-3.49609540437961));
#110309=CARTESIAN_POINT('Ctrl Pts',(-16.6336676155139,19.4761977871781,
-3.49697088317598));
#110310=CARTESIAN_POINT('Ctrl Pts',(-16.632914372631,19.4701624573689,-3.49733585020302));
#110311=CARTESIAN_POINT('Ctrl Pts',(-16.6314163088384,19.45772329401,-3.49808597904101));
#110312=CARTESIAN_POINT('Ctrl Pts',(-16.6306747091785,19.4513191306483,
-3.49847103551335));
#110313=CARTESIAN_POINT('Ctrl Pts',(-16.6290188618575,19.4364247658055,
-3.49936397324148));
#110314=CARTESIAN_POINT('Ctrl Pts',(-16.6281267018042,19.4279321833656,
-3.49987115363617));
#110315=CARTESIAN_POINT('Ctrl Pts',(-16.6254423100766,19.4008001579353,
-3.50148539257099));
#110316=CARTESIAN_POINT('Ctrl Pts',(-16.6238459509339,19.3821419125915,
-3.50258629347942));
#110317=CARTESIAN_POINT('Ctrl Pts',(-16.6207016583426,19.3385961507694,
-3.50513574072868));
#110318=CARTESIAN_POINT('Ctrl Pts',(-16.6193454211627,19.3136973424467,
-3.50657834281728));
#110319=CARTESIAN_POINT('Ctrl Pts',(-16.6161237009833,19.2260680069441,
-3.51160889038332));
#110320=CARTESIAN_POINT('Ctrl Pts',(-16.6166075134445,19.1632819493389,
-3.51512831832152));
#110321=CARTESIAN_POINT('Ctrl Pts',(-16.6250814651082,19.0009996818185,
-3.52411210307554));
#110322=CARTESIAN_POINT('Ctrl Pts',(-16.6373157489602,18.9018832699166,
-3.52948492666197));
#110323=CARTESIAN_POINT('Ctrl Pts',(-16.670520079978,18.7323939734988,-3.53889238245229));
#110324=CARTESIAN_POINT('Ctrl Pts',(-16.6882399484974,18.6615661329534,
-3.5428948538745));
#110325=CARTESIAN_POINT('Ctrl Pts',(-16.7227536191045,18.548726786343,-3.54957986307738));
#110326=CARTESIAN_POINT('Ctrl Pts',(-16.7372983176322,18.5060889678022,
-3.55218006203142));
#110327=CARTESIAN_POINT('Ctrl Pts',(-16.7558692171201,18.4568480036578,
-3.55530559412347));
#110328=CARTESIAN_POINT('Ctrl Pts',(-16.758586181469,18.4497596506939,-3.55575854114978));
#110329=CARTESIAN_POINT('Ctrl Pts',(-16.7630100799767,18.438401215764,-3.55648943866805));
#110330=CARTESIAN_POINT('Ctrl Pts',(-16.7646929344959,18.4341217424347,
-3.55676598209404));
#110331=CARTESIAN_POINT('Ctrl Pts',(-16.7677114402685,18.4265185592222,
-3.55725944103238));
#110332=CARTESIAN_POINT('Ctrl Pts',(-16.7690415984745,18.423192719539,-3.55747602418443));
#110333=CARTESIAN_POINT('Ctrl Pts',(-16.7718940390878,18.416112833291,-3.55793865400805));
#110334=CARTESIAN_POINT('Ctrl Pts',(-16.7734186337819,18.4123598335622,
-3.5581848339624));
#110335=CARTESIAN_POINT('Ctrl Pts',(-16.7775969723956,18.4021583472559,
-3.55885652889874));
#110336=CARTESIAN_POINT('Ctrl Pts',(-16.7802717936093,18.395718626447,-3.55928328913915));
#110337=CARTESIAN_POINT('Ctrl Pts',(-16.7941805734154,18.3626943136724,
-3.56148553290922));
#110338=CARTESIAN_POINT('Ctrl Pts',(-16.8059249198367,18.3363296400597,
-3.56328949110968));
#110339=CARTESIAN_POINT('Ctrl Pts',(-16.8422023566247,18.2591745322882,
-3.56868780836322));
#110340=CARTESIAN_POINT('Ctrl Pts',(-16.8682294792941,18.2091170064076,
-3.57234519506903));
#110341=CARTESIAN_POINT('Ctrl Pts',(-16.9654409722727,18.0391068316999,
-3.58517874746336));
#110342=CARTESIAN_POINT('Ctrl Pts',(-17.0464589019846,17.9251754368153,
-3.59449352641585));
#110343=CARTESIAN_POINT('Ctrl Pts',(-17.1964521749631,17.7530821288048,
-3.60922168229466));
#110344=CARTESIAN_POINT('Ctrl Pts',(-17.2589716316657,17.6898580932503,
-3.6148165912939));
#110345=CARTESIAN_POINT('Ctrl Pts',(-17.3355028063266,17.6216347455071,
-3.6210718365345));
#110346=CARTESIAN_POINT('Ctrl Pts',(-17.345807302394,17.6126266515538,-3.621902697442));
#110347=CARTESIAN_POINT('Ctrl Pts',(-17.3624837694347,17.5983311683606,
-3.62322944020701));
#110348=CARTESIAN_POINT('Ctrl Pts',(-17.3688005311341,17.5929802397703,
-3.62372794308412));
#110349=CARTESIAN_POINT('Ctrl Pts',(-17.3800785175705,17.5835397229358,
-3.62461088479693));
#110350=CARTESIAN_POINT('Ctrl Pts',(-17.3850272611905,17.579435448605,-3.6249959223352));
#110351=CARTESIAN_POINT('Ctrl Pts',(-17.3953836569019,17.5709256311373,
-3.62579676809093));
#110352=CARTESIAN_POINT('Ctrl Pts',(-17.4007945460114,17.5665241355817,
-3.62621240935285));
#110353=CARTESIAN_POINT('Ctrl Pts',(-17.4149172235604,17.5551515417235,
-3.62729013481532));
#110354=CARTESIAN_POINT('Ctrl Pts',(-17.4236626164871,17.5482223731205,
-3.62795053153846));
#110355=CARTESIAN_POINT('Ctrl Pts',(-17.462015249492,17.5183252297807,-3.63081698006998));
#110356=CARTESIAN_POINT('Ctrl Pts',(-17.4921756353886,17.4960756329734,
-3.63299460364542));
#110357=CARTESIAN_POINT('Ctrl Pts',(-17.5740157056846,17.438993369862,-3.63871976806956));
#110358=CARTESIAN_POINT('Ctrl Pts',(-17.6266702472416,17.4056211601673,
-3.64221518485314));
#110359=CARTESIAN_POINT('Ctrl Pts',(-17.762143187295,17.3279192000335,-3.65085181638876));
#110360=CARTESIAN_POINT('Ctrl Pts',(-17.846580207941,17.2866856687517,-3.65591752775121));
#110361=CARTESIAN_POINT('Ctrl Pts',(-18.0473370176224,17.2046823227886,
-3.66771458562423));
#110362=CARTESIAN_POINT('Ctrl Pts',(-18.1650196021426,17.1681908909157,
-3.67445165462703));
#110363=CARTESIAN_POINT('Ctrl Pts',(-18.2944123109063,17.1401207531809,
-3.6822994345334));
#110364=CARTESIAN_POINT('Ctrl Pts',(-18.3036548467078,17.1381803665373,
-3.68286240744297));
#110365=CARTESIAN_POINT('Ctrl Pts',(-18.3173890072432,17.1353928189708,
-3.6837029494335));
#110366=CARTESIAN_POINT('Ctrl Pts',(-18.321871037331,17.1344982286412,-3.68397788062969));
#110367=CARTESIAN_POINT('Ctrl Pts',(-18.3298599463691,17.1329305670111,
-3.68446909959897));
#110368=CARTESIAN_POINT('Ctrl Pts',(-18.333365665195,17.1322518476713,-3.68468506188026));
#110369=CARTESIAN_POINT('Ctrl Pts',(-18.3409171302157,17.1308096702755,
-3.68515113846112));
#110370=CARTESIAN_POINT('Ctrl Pts',(-18.344963332439,17.1300491545875,-3.68540141094654));
#110371=CARTESIAN_POINT('Ctrl Pts',(-18.356163642402,17.1279777757268,-3.68609563745951));
#110372=CARTESIAN_POINT('Ctrl Pts',(-18.3633222474316,17.1266919852972,
-3.68654097826476));
#110373=CARTESIAN_POINT('Ctrl Pts',(-18.4017758653499,17.1199895155955,
-3.68894141929202));
#110374=CARTESIAN_POINT('Ctrl Pts',(-18.433181384346,17.1152410370282,-3.69093103096621));
#110375=CARTESIAN_POINT('Ctrl Pts',(-18.6266011995849,17.0904330108766,
-3.70331483793629));
#110376=CARTESIAN_POINT('Ctrl Pts',(-18.7903765906892,17.0884636910055,
-3.71430960285014));
#110377=CARTESIAN_POINT('Ctrl Pts',(-19.06910665696,17.1174199346002,-3.73261520146276));
#110378=CARTESIAN_POINT('Ctrl Pts',(-19.1842754611946,17.1391327721815,
-3.74006744734212));
#110379=CARTESIAN_POINT('Ctrl Pts',(-19.3108534488288,17.1740578436693,
-3.74808511989548));
#110380=CARTESIAN_POINT('Ctrl Pts',(-19.3245916551918,17.1779985828325,
-3.74895323436935));
#110381=CARTESIAN_POINT('Ctrl Pts',(-19.3463925578859,17.1844917111299,
-3.75032772002597));
#110382=CARTESIAN_POINT('Ctrl Pts',(-19.3544815022176,17.1869537558496,
-3.75083702045052));
#110383=CARTESIAN_POINT('Ctrl Pts',(-19.3687212327373,17.1913813114083,
-3.75173244491683));
#110384=CARTESIAN_POINT('Ctrl Pts',(-19.3748781427888,17.1933266126242,
-3.75211922529926));
#110385=CARTESIAN_POINT('Ctrl Pts',(-19.3875938385896,17.1974082653848,
-3.75291728524955));
#110386=CARTESIAN_POINT('Ctrl Pts',(-19.3941512831376,17.1995485676616,
-3.75332842954848));
#110387=CARTESIAN_POINT('Ctrl Pts',(-19.4109557320203,17.2051244460932,
-3.7543810528705));
#110388=CARTESIAN_POINT('Ctrl Pts',(-19.4211871809567,17.2086065357275,
-3.75502099108923));
#110389=CARTESIAN_POINT('Ctrl Pts',(-19.4631586577787,17.2232503584544,
-3.75764265725923));
#110390=CARTESIAN_POINT('Ctrl Pts',(-19.4946581167938,17.2350899816157,
-3.75960185967755));
#110391=CARTESIAN_POINT('Ctrl Pts',(-19.5758765108759,17.2678476240938,
-3.76464255716061));
#110392=CARTESIAN_POINT('Ctrl Pts',(-19.6251029110884,17.2899238879782,
-3.76768639875721));
#110393=CARTESIAN_POINT('Ctrl Pts',(-19.787510999905,17.3703458239725,-3.77777308367551));
#110394=CARTESIAN_POINT('Ctrl Pts',(-19.8962574913671,17.4370070110241,
-3.78458681435731));
#110395=CARTESIAN_POINT('Ctrl Pts',(-20.0802516645691,17.5740147547939,
-3.79713117903374));
#110396=CARTESIAN_POINT('Ctrl Pts',(-20.1576160129603,17.6408324598594,
-3.80279979731956));
#110397=CARTESIAN_POINT('Ctrl Pts',(-20.2367056105132,17.7198062621271,
-3.80942142489032));
#110398=CARTESIAN_POINT('Ctrl Pts',(-20.2435159628775,17.7267006819732,
-3.8099989237236));
#110399=CARTESIAN_POINT('Ctrl Pts',(-20.2535018100779,17.7369495999,-3.81085701749585));
#110400=CARTESIAN_POINT('Ctrl Pts',(-20.256714157878,17.740268234743,-3.81113481182217));
#110401=CARTESIAN_POINT('Ctrl Pts',(-20.2623940492995,17.7461746126948,
-3.81162917255182));
#110402=CARTESIAN_POINT('Ctrl Pts',(-20.2648659241496,17.7487581228484,
-3.81184539723922));
#110403=CARTESIAN_POINT('Ctrl Pts',(-20.2701482858008,17.7543071234984,
-3.81230980404747));
#110404=CARTESIAN_POINT('Ctrl Pts',(-20.2729566942511,17.7572744464699,
-3.81255813260732));
#110405=CARTESIAN_POINT('Ctrl Pts',(-20.2787023604173,17.7633805412943,
-3.81306907659211));
#110406=CARTESIAN_POINT('Ctrl Pts',(-20.2816386810215,17.7665201656755,
-3.8133317601623));
#110407=CARTESIAN_POINT('Ctrl Pts',(-20.2950923997718,17.780993500406,-3.81454245989279));
#110408=CARTESIAN_POINT('Ctrl Pts',(-20.3054946781769,17.7924329363557,
-3.81549868737895));
#110409=CARTESIAN_POINT('Ctrl Pts',(-20.3738026541683,17.8692249566307,
-3.82190713037721));
#110410=CARTESIAN_POINT('Ctrl Pts',(-20.4277374315831,17.9379864932015,
-3.82759173623723));
#110411=CARTESIAN_POINT('Ctrl Pts',(-20.5185485967195,18.0697861553104,
-3.83812738061853));
#110412=CARTESIAN_POINT('Ctrl Pts',(-20.5567134709897,18.131788025879,-3.84295322228073));
#110413=CARTESIAN_POINT('Ctrl Pts',(-20.5938938258958,18.199809306751,-3.84805125631605));
#110414=CARTESIAN_POINT('Ctrl Pts',(-20.5961629620878,18.2039941586156,
-3.84836414488516));
#110415=CARTESIAN_POINT('Ctrl Pts',(-20.6463823918028,18.2973614898272,
-3.85532785540514));
#110416=CARTESIAN_POINT('Ctrl Pts',(-20.6878719037659,18.3898338429119,
-3.86186883282244));
#110417=CARTESIAN_POINT('Ctrl Pts',(-20.7225805460717,18.4848895319684,
-3.86819362763421));
#110418=CARTESIAN_POINT('',(-20.8509991606888,19.2128851108726,-2.8890562790225));
#110419=CARTESIAN_POINT('Ctrl Pts',(-20.7225806137986,18.4848897174502,
-3.64442447432525));
#110420=CARTESIAN_POINT('Ctrl Pts',(-20.697586191156,18.4164380985782,-3.64005128981157));
#110421=CARTESIAN_POINT('Ctrl Pts',(-20.6690382458922,18.3492373239759,
-3.6356781052979));
#110422=CARTESIAN_POINT('Ctrl Pts',(-20.6370917888833,18.2836755459468,
-3.63130492078422));
#110423=CARTESIAN_POINT('Ctrl Pts',(-20.6051516528636,18.2181267401009,
-3.62693260155749));
#110424=CARTESIAN_POINT('Ctrl Pts',(-20.5698145519931,18.1542167202052,
-3.62256028233075));
#110425=CARTESIAN_POINT('Ctrl Pts',(-20.5312826515011,18.0923114505756,
-3.61818796310402));
#110426=CARTESIAN_POINT('Ctrl Pts',(-20.4927456644625,18.030398008911,-3.61381506669306));
#110427=CARTESIAN_POINT('Ctrl Pts',(-20.4510132974867,17.9704902511049,
-3.60944217028209));
#110428=CARTESIAN_POINT('Ctrl Pts',(-20.4063315674442,17.9129259926608,
-3.60506927387112));
#110429=CARTESIAN_POINT('Ctrl Pts',(-20.3616005534068,17.8552982407795,
-3.60069155415084));
#110430=CARTESIAN_POINT('Ctrl Pts',(-20.313913981681,17.8000195274286,-3.59631383443056));
#110431=CARTESIAN_POINT('Ctrl Pts',(-20.2635582109227,17.7473946298954,
-3.59193611471028));
#110432=CARTESIAN_POINT('Ctrl Pts',(-20.2131701327735,17.694735969139,-3.58755558632081));
#110433=CARTESIAN_POINT('Ctrl Pts',(-20.1601097989142,17.6447348427113,
-3.58317505793135));
#110434=CARTESIAN_POINT('Ctrl Pts',(-20.1046985222746,17.5976573330398,
-3.57879452954188));
#110435=CARTESIAN_POINT('Ctrl Pts',(-20.049194460902,17.55050099331,-3.57440666607223));
#110436=CARTESIAN_POINT('Ctrl Pts',(-19.9913319847969,17.5062783305872,
-3.57001880260258));
#110437=CARTESIAN_POINT('Ctrl Pts',(-19.931462691737,17.4652130422363,-3.56563093913294));
#110438=CARTESIAN_POINT('Ctrl Pts',(-19.9100486473828,17.4505248129083,
-3.56406148844868));
#110439=CARTESIAN_POINT('Ctrl Pts',(-19.8883780972448,17.4362400977019,
-3.56249203776441));
#110440=CARTESIAN_POINT('Ctrl Pts',(-19.8664678605235,17.4223676887405,
-3.56092258708015));
#110441=CARTESIAN_POINT('Ctrl Pts',(-19.8052064921928,17.3835802139256,
-3.55653437814987));
#110442=CARTESIAN_POINT('Ctrl Pts',(-19.7418305075797,17.3478680068776,
-3.55214616921958));
#110443=CARTESIAN_POINT('Ctrl Pts',(-19.6766813842658,17.3154681992225,
-3.54775796028929));
#110444=CARTESIAN_POINT('Ctrl Pts',(-19.6116289530529,17.2831164782541,
-3.54337626418865));
#110445=CARTESIAN_POINT('Ctrl Pts',(-19.5448090356316,17.254067610473,-3.538994568088));
#110446=CARTESIAN_POINT('Ctrl Pts',(-19.4765908557835,17.22851473627,-3.53461287198736));
#110447=CARTESIAN_POINT('Ctrl Pts',(-19.4084528377258,17.2029918887278,
-3.53023632472834));
#110448=CARTESIAN_POINT('Ctrl Pts',(-19.3389202706951,17.180957042421,-3.52585977746933));
#110449=CARTESIAN_POINT('Ctrl Pts',(-19.2683841301345,17.1625560536201,
-3.52148323021032));
#110450=CARTESIAN_POINT('Ctrl Pts',(-19.1978927225693,17.144166734459,-3.51710945849398));
#110451=CARTESIAN_POINT('Ctrl Pts',(-19.1263994698853,17.129406821763,-3.51273568677764));
#110452=CARTESIAN_POINT('Ctrl Pts',(-19.0543110010047,17.1183724978785,
-3.50836191506129));
#110453=CARTESIAN_POINT('Ctrl Pts',(-18.9822444688873,17.1073415317758,
-3.50398947429838));
#110454=CARTESIAN_POINT('Ctrl Pts',(-18.9095835567026,17.1000339766643,
-3.49961703353547));
#110455=CARTESIAN_POINT('Ctrl Pts',(-18.8367439345939,17.0964946952291,
-3.49524459277255));
#110456=CARTESIAN_POINT('Ctrl Pts',(-18.7639024499681,17.0929553232941,
-3.49087204020585));
#110457=CARTESIAN_POINT('Ctrl Pts',(-18.6908827282521,17.0931844377534,
-3.48649948763914));
#110458=CARTESIAN_POINT('Ctrl Pts',(-18.6181027067728,17.0971748375463,
-3.48212693507243));
#110459=CARTESIAN_POINT('Ctrl Pts',(-18.5452471514419,17.1011693787266,
-3.47774984450575));
#110460=CARTESIAN_POINT('Ctrl Pts',(-18.4726322757184,17.1089329725838,
-3.47337275393906));
#110461=CARTESIAN_POINT('Ctrl Pts',(-18.4006723159502,17.1204063869212,
-3.46899566337237));
#110462=CARTESIAN_POINT('Ctrl Pts',(-18.3286730561771,17.1318860673159,
-3.46461618231407));
#110463=CARTESIAN_POINT('Ctrl Pts',(-18.257329896609,17.1470795015326,-3.46023670125577));
#110464=CARTESIAN_POINT('Ctrl Pts',(-18.1870456019972,17.1658765595922,
-3.45585722019747));
#110465=CARTESIAN_POINT('Ctrl Pts',(-18.1166367289449,17.1847069353111,
-3.45146997653838));
#110466=CARTESIAN_POINT('Ctrl Pts',(-18.0472909281422,17.2071535415658,
-3.4470827328793));
#110467=CARTESIAN_POINT('Ctrl Pts',(-17.9793940004948,17.23305693067,-3.44269548922021));
#110468=CARTESIAN_POINT('Ctrl Pts',(-17.9332306321323,17.2506687392522,
-3.43971258627972));
#110469=CARTESIAN_POINT('Ctrl Pts',(-17.8877366290248,17.2698774944525,
-3.43672968333922));
#110470=CARTESIAN_POINT('Ctrl Pts',(-17.8430266573744,17.290621000237,-3.43374678039872));
#110471=CARTESIAN_POINT('Ctrl Pts',(-17.7772529124843,17.3211371917539,
-3.42935857146461));
#110472=CARTESIAN_POINT('Ctrl Pts',(-17.7129203794319,17.3550960250395,
-3.4249703625305));
#110473=CARTESIAN_POINT('Ctrl Pts',(-17.6504132837264,17.3923387263387,
-3.42058215359639));
#110474=CARTESIAN_POINT('Ctrl Pts',(-17.5879989589145,17.4295261532943,
-3.4162004574919));
#110475=CARTESIAN_POINT('Ctrl Pts',(-17.5274051041883,17.469987528232,-3.41181876138741));
#110476=CARTESIAN_POINT('Ctrl Pts',(-17.4689939738816,17.5135169356119,
-3.40743706528292));
#110477=CARTESIAN_POINT('Ctrl Pts',(-17.4106514813017,17.556995192474,-3.40306051802006));
#110478=CARTESIAN_POINT('Ctrl Pts',(-17.354487002868,17.6035340332478,-3.3986839707572));
#110479=CARTESIAN_POINT('Ctrl Pts',(-17.3008348082142,17.6528836586912,
-3.39430742349434));
#110480=CARTESIAN_POINT('Ctrl Pts',(-17.2472166390025,17.7022019873193,
-3.38993365177416));
#110481=CARTESIAN_POINT('Ctrl Pts',(-17.1961079465059,17.7543272380327,
-3.38555988005397));
#110482=CARTESIAN_POINT('Ctrl Pts',(-17.14780970538,17.8089695619377,-3.38118610833378));
#110483=CARTESIAN_POINT('Ctrl Pts',(-17.099526161571,17.8635952579999,-3.37681366756702));
#110484=CARTESIAN_POINT('Ctrl Pts',(-17.0540516905114,17.9207361453885,
-3.37244122680026));
#110485=CARTESIAN_POINT('Ctrl Pts',(-17.0116490089847,17.980066994614,-3.3680687860335));
#110486=CARTESIAN_POINT('Ctrl Pts',(-16.9692452432169,18.0393993609357,
-3.36369623346297));
#110487=CARTESIAN_POINT('Ctrl Pts',(-16.92991370178,18.100921406656,-3.35932368089243));
#110488=CARTESIAN_POINT('Ctrl Pts',(-16.8938745512702,18.1642778148253,
-3.3549511283219));
#110489=CARTESIAN_POINT('Ctrl Pts',(-16.857797997971,18.227699976664,-3.35057403775142));
#110490=CARTESIAN_POINT('Ctrl Pts',(-16.82502089682,18.2929598817714,-3.34619694718094));
#110491=CARTESIAN_POINT('Ctrl Pts',(-16.7957176611922,18.3596771616679,
-3.34181985661046));
#110492=CARTESIAN_POINT('Ctrl Pts',(-16.76639842198,18.4264308783469,-3.33744037554839));
#110493=CARTESIAN_POINT('Ctrl Pts',(-16.7405569966208,18.4946431030916,
-3.33306089448631));
#110494=CARTESIAN_POINT('Ctrl Pts',(-16.718318792152,18.5639155632158,-3.32868141342424));
#110495=CARTESIAN_POINT('Ctrl Pts',(-16.6960411706153,18.6333108083096,
-3.32429416976145));
#110496=CARTESIAN_POINT('Ctrl Pts',(-16.6773796475306,18.7037695748786,
-3.31990692609866));
#110497=CARTESIAN_POINT('Ctrl Pts',(-16.6624089793399,18.7748811594065,
-3.31551968243587));
#110498=CARTESIAN_POINT('Ctrl Pts',(-16.6522303676452,18.8232301840919,
-3.31253677952968));
#110499=CARTESIAN_POINT('Ctrl Pts',(-16.6437568500118,18.8718807754355,
-3.30955387662348));
#110500=CARTESIAN_POINT('Ctrl Pts',(-16.6369981960583,18.920702851779,-3.30657097371728));
#110501=CARTESIAN_POINT('Ctrl Pts',(-16.6270554032346,18.9925259978739,
-3.30218276479083));
#110502=CARTESIAN_POINT('Ctrl Pts',(-16.6207874279489,19.0650007495852,
-3.29779455586437));
#110503=CARTESIAN_POINT('Ctrl Pts',(-16.6182687405808,19.1377180928438,
-3.29340634693792));
#110504=CARTESIAN_POINT('Ctrl Pts',(-16.6157537913624,19.2103275115083,
-3.28902465084108));
#110505=CARTESIAN_POINT('Ctrl Pts',(-16.6169771002007,19.2831783288758,
-3.28464295474424));
#110506=CARTESIAN_POINT('Ctrl Pts',(-16.6219616061144,19.3558544882043,
-3.2802612586474));
#110507=CARTESIAN_POINT('Ctrl Pts',(-16.6269402548369,19.4284452472623,
-3.27588471139215));
#110508=CARTESIAN_POINT('Ctrl Pts',(-16.6356712880179,19.5008612771275,
-3.27150816413689));
#110509=CARTESIAN_POINT('Ctrl Pts',(-16.6481255978395,19.5726862983464,
-3.26713161688164));
#110510=CARTESIAN_POINT('Ctrl Pts',(-16.6605720093188,19.6444657691812,
-3.26275784516903));
#110511=CARTESIAN_POINT('Ctrl Pts',(-16.6767369302058,19.7156545009234,
-3.25838407345642));
#110512=CARTESIAN_POINT('Ctrl Pts',(-16.6965395553233,19.7858425318102,
-3.2540103017438));
#110513=CARTESIAN_POINT('Ctrl Pts',(-16.7163361544357,19.8560092042441,
-3.24963786098458));
#110514=CARTESIAN_POINT('Ctrl Pts',(-16.7397681292064,19.9251753164071,
-3.24526542022535));
#110515=CARTESIAN_POINT('Ctrl Pts',(-16.766704216716,19.9929439245068,-3.24089297946613));
#110516=CARTESIAN_POINT('Ctrl Pts',(-16.7936409929846,20.0607142654578,
-3.23652042690307));
#110517=CARTESIAN_POINT('Ctrl Pts',(-16.8240818798544,20.1270865838709,
-3.23214787434001));
#110518=CARTESIAN_POINT('Ctrl Pts',(-16.8578472840037,20.1916834281559,
-3.22777532177696));
#110519=CARTESIAN_POINT('Ctrl Pts',(-16.8916477311638,20.2563473134839,
-3.22339823121383));
#110520=CARTESIAN_POINT('Ctrl Pts',(-16.9287793604432,20.3192316172878,
-3.2190211406507));
#110521=CARTESIAN_POINT('Ctrl Pts',(-16.9690167487975,20.3799837992782,
-3.21464405008757));
#110522=CARTESIAN_POINT('Ctrl Pts',(-17.0092761122835,20.4407691602906,
-3.21026456903279));
#110523=CARTESIAN_POINT('Ctrl Pts',(-17.0526443249069,20.4994196929899,
-3.205885087978));
#110524=CARTESIAN_POINT('Ctrl Pts',(-17.0988543828178,20.555614372454,-3.20150560692321));
#110525=CARTESIAN_POINT('Ctrl Pts',(-17.1451463477475,20.6119086566118,
-3.19711836326753));
#110526=CARTESIAN_POINT('Ctrl Pts',(-17.1942898914314,20.6657380382439,
-3.19273111961185));
#110527=CARTESIAN_POINT('Ctrl Pts',(-17.2459801414521,20.7168173529904,
-3.18834387595617));
#110528=CARTESIAN_POINT('Ctrl Pts',(-17.281124531093,20.7515463655087,-3.18536097298273));
#110529=CARTESIAN_POINT('Ctrl Pts',(-17.3174454256988,20.7850048960141,
-3.18237807000929));
#110530=CARTESIAN_POINT('Ctrl Pts',(-17.3548387352823,20.8171143190639,
-3.17939516703585));
#110531=CARTESIAN_POINT('Ctrl Pts',(-17.4098487897264,20.8643511411001,
-3.17500695810762));
#110532=CARTESIAN_POINT('Ctrl Pts',(-17.4673958504113,20.9088507249,-3.1706187491794));
#110533=CARTESIAN_POINT('Ctrl Pts',(-17.5271763106369,20.9503290611015,
-3.16623054025117));
#110534=CARTESIAN_POINT('Ctrl Pts',(-17.5868680467469,20.9917458365741,
-3.16184884415263));
#110535=CARTESIAN_POINT('Ctrl Pts',(-17.6487862091497,21.0301499931519,
-3.15746714805409));
#110536=CARTESIAN_POINT('Ctrl Pts',(-17.7125933764233,21.0652970391266,
-3.15308545195556));
#110537=CARTESIAN_POINT('Ctrl Pts',(-17.7763255651964,21.1004027845246,
-3.14870890469871));
#110538=CARTESIAN_POINT('Ctrl Pts',(-17.8419419289088,21.1322587908217,
-3.14433235744187));
#110539=CARTESIAN_POINT('Ctrl Pts',(-17.9090766869082,21.1606642089133,
-3.13995581018503));
#110540=CARTESIAN_POINT('Ctrl Pts',(-17.9761688690191,21.1890516127013,
-3.1355820384709));
#110541=CARTESIAN_POINT('Ctrl Pts',(-18.044777091656,21.2139925826767,-3.13120826675677));
#110542=CARTESIAN_POINT('Ctrl Pts',(-18.1145129035447,21.2353331586785,
-3.12683449504263));
#110543=CARTESIAN_POINT('Ctrl Pts',(-18.1842274945909,21.2566672406712,
-3.12246205428196));
#110544=CARTESIAN_POINT('Ctrl Pts',(-18.2550685326861,21.2744029627471,
-3.11808961352129));
#110545=CARTESIAN_POINT('Ctrl Pts',(-18.3266312007897,21.2884358381019,
-3.11371717276062));
#110546=CARTESIAN_POINT('Ctrl Pts',(-18.3981956987582,21.3024690722787,
-3.10934462019619));
#110547=CARTESIAN_POINT('Ctrl Pts',(-18.4704813896227,21.3127991808916,
-3.10497206763176));
#110548=CARTESIAN_POINT('Ctrl Pts',(-18.5430736858703,21.3193728661157,
-3.10059951506733));
#110549=CARTESIAN_POINT('Ctrl Pts',(-18.6157413211406,21.3259533737582,
-3.09622242450294));
#110550=CARTESIAN_POINT('Ctrl Pts',(-18.6887157156752,21.3287696306809,
-3.09184533393856));
#110551=CARTESIAN_POINT('Ctrl Pts',(-18.7615784216629,21.3278203586177,
-3.08746824337417));
#110552=CARTESIAN_POINT('Ctrl Pts',(-18.8344809206782,21.3268705681219,
-3.0830887623182));
#110553=CARTESIAN_POINT('Ctrl Pts',(-18.9072711280009,21.3221511854097,
-3.07870928126222));
#110554=CARTESIAN_POINT('Ctrl Pts',(-18.9795345883547,21.3137129537627,
-3.07432980020625));
#110555=CARTESIAN_POINT('Ctrl Pts',(-19.0519261352069,21.3052597654067,
-3.06994255654949));
#110556=CARTESIAN_POINT('Ctrl Pts',(-19.12378859461,21.2930746456018,-3.06555531289274));
#110557=CARTESIAN_POINT('Ctrl Pts',(-19.1947171668079,21.2772595897439,
-3.06116806923599));
#110558=CARTESIAN_POINT('Ctrl Pts',(-19.2429417616898,21.2665068755957,
-3.05818516627546));
#110559=CARTESIAN_POINT('Ctrl Pts',(-19.2907349020845,21.2540772191552,
-3.05520226331494));
#110560=CARTESIAN_POINT('Ctrl Pts',(-19.3379741345029,21.2400155851672,
-3.05221936035441));
#110561=CARTESIAN_POINT('Ctrl Pts',(-19.4074687259705,21.2193292306409,
-3.04783115140145));
#110562=CARTESIAN_POINT('Ctrl Pts',(-19.476034966597,21.195028040176,-3.04344294244849));
#110563=CARTESIAN_POINT('Ctrl Pts',(-19.5432697129023,21.1672135700835,
-3.03905473349553));
#110564=CARTESIAN_POINT('Ctrl Pts',(-19.610404671698,21.1394403812758,-3.03467303737213));
#110565=CARTESIAN_POINT('Ctrl Pts',(-19.6762116170599,21.1081644467917,
-3.03029134124872));
#110566=CARTESIAN_POINT('Ctrl Pts',(-19.7403023303344,21.0735371459285,
-3.02590964512532));
#110567=CARTESIAN_POINT('Ctrl Pts',(-19.8043177319206,21.0389505348994,
-3.02153309784355));
#110568=CARTESIAN_POINT('Ctrl Pts',(-19.8666204853357,21.0010206087535,
-3.01715655056178));
#110569=CARTESIAN_POINT('Ctrl Pts',(-19.926843718136,20.9599462153261,-3.01278000328));
#110570=CARTESIAN_POINT('Ctrl Pts',(-19.9870287582372,20.9188978706821,
-3.00840623154091));
#110571=CARTESIAN_POINT('Ctrl Pts',(-20.0451364968644,20.874709286591,-3.00403245980182));
#110572=CARTESIAN_POINT('Ctrl Pts',(-20.1008272165774,20.8276237533896,
-2.99965868806273));
#110573=CARTESIAN_POINT('Ctrl Pts',(-20.1565009894169,20.7805525484744,
-2.9952862472771));
#110574=CARTESIAN_POINT('Ctrl Pts',(-20.2097588354092,20.7305864558568,
-2.99091380649147));
#110575=CARTESIAN_POINT('Ctrl Pts',(-20.2602937778995,20.6780093058823,
-2.98654136570585));
#110576=CARTESIAN_POINT('Ctrl Pts',(-20.3108300125729,20.6254308115053,
-2.9821688131165));
#110577=CARTESIAN_POINT('Ctrl Pts',(-20.3586428726808,20.5702414763812,
-2.97779626052716));
#110578=CARTESIAN_POINT('Ctrl Pts',(-20.4034631348275,20.5127610539004,
-2.97342370793782));
#110579=CARTESIAN_POINT('Ctrl Pts',(-20.4483299131299,20.4552209760729,
-2.96904661734876));
#110580=CARTESIAN_POINT('Ctrl Pts',(-20.4901975952178,20.3953854447133,
-2.9646695267597));
#110581=CARTESIAN_POINT('Ctrl Pts',(-20.5288386084058,20.3336056163123,
-2.96029243617064));
#110582=CARTESIAN_POINT('Ctrl Pts',(-20.5675007248842,20.2717920476558,
-2.95591295509008));
#110583=CARTESIAN_POINT('Ctrl Pts',(-20.6029324294579,20.2080324897585,
-2.95153347400953));
#110584=CARTESIAN_POINT('Ctrl Pts',(-20.6349520524139,20.1427029002979,
-2.94715399292897));
#110585=CARTESIAN_POINT('Ctrl Pts',(-20.6670284299332,20.0772575145854,
-2.94276674924806));
#110586=CARTESIAN_POINT('Ctrl Pts',(-20.6956804586539,20.0102369839667,
-2.93837950556715));
#110587=CARTESIAN_POINT('Ctrl Pts',(-20.7207747901306,19.9420368891524,
-2.93399226188624));
#110588=CARTESIAN_POINT('Ctrl Pts',(-20.7378365162411,19.8956673997114,
-2.93100935914849));
#110589=CARTESIAN_POINT('Ctrl Pts',(-20.7532546613793,19.8487529982427,
-2.92802645641074));
#110590=CARTESIAN_POINT('Ctrl Pts',(-20.7670007520344,19.8014209872857,
-2.92504355367298));
#110591=CARTESIAN_POINT('Ctrl Pts',(-20.7921933233445,19.7146752287136,
-2.9195767637458));
#110592=CARTESIAN_POINT('Ctrl Pts',(-20.8118478930297,19.6262535084729,
-2.91410997381861));
#110593=CARTESIAN_POINT('Ctrl Pts',(-20.8257819138181,19.5367873923641,
-2.90864318389142));
#110594=CARTESIAN_POINT('Ctrl Pts',(-20.8394880731092,19.448784305735,-2.90326579177394));
#110595=CARTESIAN_POINT('Ctrl Pts',(-20.8476592207556,19.359770608721,-2.89788839965646));
#110596=CARTESIAN_POINT('Ctrl Pts',(-20.8501673751636,19.2703686810797,
-2.89251100753897));
#110597=CARTESIAN_POINT('Ctrl Pts',(-20.8507044999983,19.2512231310868,
-2.89135943136681));
#110598=CARTESIAN_POINT('Ctrl Pts',(-20.8509820862726,19.2320598582094,
-2.89020785519466));
#110599=CARTESIAN_POINT('Ctrl Pts',(-20.8509991606888,19.2128851108726,
-2.8890562790225));
#110600=CARTESIAN_POINT('Ctrl Pts',(-20.8499621049652,19.2128841874121,
-2.8890562790225));
#110601=CARTESIAN_POINT('Ctrl Pts',(-20.8478499548941,18.9660537307247,
-2.87422526267969));
#110602=CARTESIAN_POINT('Ctrl Pts',(-20.8034780943232,18.7185580611686,
-2.85939424633688));
#110603=CARTESIAN_POINT('Ctrl Pts',(-20.7202231698227,18.4857291668958,
-2.84456322999407));
#110604=CARTESIAN_POINT('Origin',(-18.734,19.211,0.));
#110605=CARTESIAN_POINT('',(-20.7225806143688,18.484889719012,-2.04625075898636));
#110606=CARTESIAN_POINT('',(-20.7225806137756,18.4848897173872,-2.26547387919804));
#110607=CARTESIAN_POINT('',(-20.7225806137986,18.4848897174502,0.));
#110608=CARTESIAN_POINT('',(-20.8509992561162,19.2092252878304,-2.31031848245491));
#110609=CARTESIAN_POINT('Ctrl Pts',(-20.7225806137756,18.4848897173872,
-2.26547387919804));
#110610=CARTESIAN_POINT('Ctrl Pts',(-20.7575267776174,18.5805959284211,
-2.27104577281407));
#110611=CARTESIAN_POINT('Ctrl Pts',(-20.7855141372301,18.6786892936843,
-2.27670321222546));
#110612=CARTESIAN_POINT('Ctrl Pts',(-20.8083091756226,18.7878873309347,
-2.28331207106325));
#110613=CARTESIAN_POINT('Ctrl Pts',(-20.8102239921009,18.7973856707489,
-2.28388948204838));
#110614=CARTESIAN_POINT('Ctrl Pts',(-20.8129550905691,18.8114301543172,
-2.28474746974855));
#110615=CARTESIAN_POINT('Ctrl Pts',(-20.8138218376122,18.81596651655,-2.28502524684811));
#110616=CARTESIAN_POINT('Ctrl Pts',(-20.8153332691877,18.8240198873561,
-2.28551958855298));
#110617=CARTESIAN_POINT('Ctrl Pts',(-20.8159838950629,18.8275357311319,
-2.28573581153983));
#110618=CARTESIAN_POINT('Ctrl Pts',(-20.8173589186186,18.835072732932,-2.28620022787933));
#110619=CARTESIAN_POINT('Ctrl Pts',(-20.8180805722734,18.8390942840813,
-2.28644856773996));
#110620=CARTESIAN_POINT('Ctrl Pts',(-20.8195376389239,18.8473514906243,
-2.28695953916183));
#110621=CARTESIAN_POINT('Ctrl Pts',(-20.8202718002692,18.8515873452387,
-2.28722223889673));
#110622=CARTESIAN_POINT('Ctrl Pts',(-20.8220971197962,18.8623128553873,
-2.28788882365087));
#110623=CARTESIAN_POINT('Ctrl Pts',(-20.8231709205875,18.8688053645306,
-2.28829363336577));
#110624=CARTESIAN_POINT('Ctrl Pts',(-20.8419517333687,18.9857438180572,
-2.29560693393806));
#110625=CARTESIAN_POINT('Ctrl Pts',(-20.8509055124976,19.09740142457,-2.30293673158685));
#110626=CARTESIAN_POINT('Ctrl Pts',(-20.8509992561162,19.2092252878304,
-2.31031848245491));
#110627=CARTESIAN_POINT('Ctrl Pts',(-20.8509992546752,19.2092235697065,
-2.3103183690376));
#110628=CARTESIAN_POINT('Ctrl Pts',(-20.8510842733415,19.3105416195705,
-2.31700660648527));
#110629=CARTESIAN_POINT('Ctrl Pts',(-20.8438956122245,19.411744162389,-2.32371997042176));
#110630=CARTESIAN_POINT('Ctrl Pts',(-20.816945499949,19.5993334523545,-2.3359902690649));
#110631=CARTESIAN_POINT('Ctrl Pts',(-20.7989633480779,19.68575741357,-2.34157368887109));
#110632=CARTESIAN_POINT('Ctrl Pts',(-20.7702151430968,19.7906013393171,
-2.34824550970317));
#110633=CARTESIAN_POINT('Ctrl Pts',(-20.7645030413533,19.8103056541231,
-2.34949516767977));
#110634=CARTESIAN_POINT('Ctrl Pts',(-20.7559151380913,19.8383967355679,
-2.35127116134167));
#110635=CARTESIAN_POINT('Ctrl Pts',(-20.7532718148567,19.8468528374542,
-2.35180505435446));
#110636=CARTESIAN_POINT('Ctrl Pts',(-20.7485973731832,19.8614834109189,
-2.35272759918289));
#110637=CARTESIAN_POINT('Ctrl Pts',(-20.7465907736203,19.8676655338283,
-2.35311705013428));
#110638=CARTESIAN_POINT('Ctrl Pts',(-20.7426778410658,19.8795344437417,
-2.35386407396392));
#110639=CARTESIAN_POINT('Ctrl Pts',(-20.7407757522852,19.8852225543821,
-2.35422178228765));
#110640=CARTESIAN_POINT('Ctrl Pts',(-20.7357295714573,19.9001023825438,
-2.35515678928988));
#110641=CARTESIAN_POINT('Ctrl Pts',(-20.7325463160518,19.9092807445782,
-2.35573278836707));
#110642=CARTESIAN_POINT('Ctrl Pts',(-20.7212792307712,19.9410591434125,
-2.35772476148054));
#110643=CARTESIAN_POINT('Ctrl Pts',(-20.7128741355498,19.9635438981978,
-2.35913006618206));
#110644=CARTESIAN_POINT('Ctrl Pts',(-20.6487986693639,20.1264517915341,
-2.3692920817944));
#110645=CARTESIAN_POINT('Ctrl Pts',(-20.5786228615951,20.2607043462482,
-2.37751642346493));
#110646=CARTESIAN_POINT('Ctrl Pts',(-20.4575557914712,20.4420692461861,
-2.38935813821247));
#110647=CARTESIAN_POINT('Ctrl Pts',(-20.4177432945758,20.4959840616474,
-2.39299178975612));
#110648=CARTESIAN_POINT('Ctrl Pts',(-20.3413736394659,20.5897492521361,
-2.3996784945855));
#110649=CARTESIAN_POINT('Ctrl Pts',(-20.3057195788503,20.6302590608486,
-2.40270481271704));
#110650=CARTESIAN_POINT('Ctrl Pts',(-20.2493176372455,20.6896080313168,
-2.40743005519066));
#110651=CARTESIAN_POINT('Ctrl Pts',(-20.2296773230086,20.7094720308871,
-2.40906500584354));
#110652=CARTESIAN_POINT('Ctrl Pts',(-20.2047675557869,20.7336878144113,
-2.41113482568634));
#110653=CARTESIAN_POINT('Ctrl Pts',(-20.1998614359622,20.7384114151063,
-2.41154231133627));
#110654=CARTESIAN_POINT('Ctrl Pts',(-20.1919761568931,20.7459303615268,
-2.41219712197122));
#110655=CARTESIAN_POINT('Ctrl Pts',(-20.189011503163,20.7487409449644,-2.41244328774043));
#110656=CARTESIAN_POINT('Ctrl Pts',(-20.1834366926422,20.7539954827986,
-2.41290617899004));
#110657=CARTESIAN_POINT('Ctrl Pts',(-20.1808284727663,20.7564414112569,
-2.41312274826207));
#110658=CARTESIAN_POINT('Ctrl Pts',(-20.17483648468,20.7620320963126,-2.41362027704958));
#110659=CARTESIAN_POINT('Ctrl Pts',(-20.1714486213068,20.7651723841151,
-2.41390157141762));
#110660=CARTESIAN_POINT('Ctrl Pts',(-20.1609189967142,20.7748686527225,
-2.41477574451773));
#110661=CARTESIAN_POINT('Ctrl Pts',(-20.153742577207,20.7813865741958,-2.4153713888015));
#110662=CARTESIAN_POINT('Ctrl Pts',(-20.0721339819135,20.8544902726283,
-2.42214070564147));
#110663=CARTESIAN_POINT('Ctrl Pts',(-19.993132486254,20.9157707986147,-2.42864913286996));
#110664=CARTESIAN_POINT('Ctrl Pts',(-19.7683137215159,21.065984540022,-2.44646383483442));
#110665=CARTESIAN_POINT('Ctrl Pts',(-19.6155580137379,21.1432644447314,
-2.45778783330393));
#110666=CARTESIAN_POINT('Ctrl Pts',(-19.4275334683066,21.2113910572846,
-2.47032159553595));
#110667=CARTESIAN_POINT('Ctrl Pts',(-19.3996902815741,21.2208282605146,
-2.47214593254641));
#110668=CARTESIAN_POINT('Ctrl Pts',(-19.3513347991858,21.2361027161312,
-2.47526061096035));
#110669=CARTESIAN_POINT('Ctrl Pts',(-19.3309147912726,21.2422154118328,
-2.47655968214315));
#110670=CARTESIAN_POINT('Ctrl Pts',(-19.3017486516981,21.2504684128913,
-2.47839278320209));
#110671=CARTESIAN_POINT('Ctrl Pts',(-19.2930763246305,21.2528627784035,
-2.47893505333509));
#110672=CARTESIAN_POINT('Ctrl Pts',(-19.2780892874396,21.2568979469085,
-2.47986744792713));
#110673=CARTESIAN_POINT('Ctrl Pts',(-19.2717818225323,21.258564962267,-2.48025841872149));
#110674=CARTESIAN_POINT('Ctrl Pts',(-19.2596903612465,21.2617009178522,
-2.48100519921622));
#110675=CARTESIAN_POINT('Ctrl Pts',(-19.2539076720035,21.2631746085804,
-2.48136115945331));
#110676=CARTESIAN_POINT('Ctrl Pts',(-19.23885498646,21.2669430048263,-2.48228471066503));
#110677=CARTESIAN_POINT('Ctrl Pts',(-19.2295754908998,21.2691994883416,
-2.48285106439092));
#110678=CARTESIAN_POINT('Ctrl Pts',(-19.1978835578883,21.2766792174888,
-2.48477539785402));
#110679=CARTESIAN_POINT('Ctrl Pts',(-19.1754008740866,21.2815998923722,
-2.48612366778171));
#110680=CARTESIAN_POINT('Ctrl Pts',(-18.9811155913145,21.3208137639462,
-2.49764070408457));
#110681=CARTESIAN_POINT('Ctrl Pts',(-18.8057534490266,21.3340257628163,
-2.50706151055773));
#110682=CARTESIAN_POINT('Ctrl Pts',(-18.5436506241012,21.3212277460492,
-2.52133910042804));
#110683=CARTESIAN_POINT('Ctrl Pts',(-18.4569002396963,21.3115969010905,
-2.5261126611607));
#110684=CARTESIAN_POINT('Ctrl Pts',(-18.3336850957124,21.2901516186535,
-2.53325294949115));
#110685=CARTESIAN_POINT('Ctrl Pts',(-18.2965551366273,21.2826575650292,
-2.53545288700559));
#110686=CARTESIAN_POINT('Ctrl Pts',(-18.2522667891114,21.2724750759142,
-2.53815665528862));
#110687=CARTESIAN_POINT('Ctrl Pts',(-18.2448940388325,21.2707382673315,
-2.53860943002565));
#110688=CARTESIAN_POINT('Ctrl Pts',(-18.2334646416941,21.2679810042325,
-2.53931571147065));
#110689=CARTESIAN_POINT('Ctrl Pts',(-18.2294013452952,21.2669880091243,
-2.53956766525062));
#110690=CARTESIAN_POINT('Ctrl Pts',(-18.2218817238485,21.2651267174715,
-2.54003557824757));
#110691=CARTESIAN_POINT('Ctrl Pts',(-18.2184246383238,21.26426173345,-2.54025134535867));
#110692=CARTESIAN_POINT('Ctrl Pts',(-18.2106271651465,21.2622898234599,
-2.54073946802716));
#110693=CARTESIAN_POINT('Ctrl Pts',(-18.2062881220939,21.2611778550058,
-2.54101211035463));
#110694=CARTESIAN_POINT('Ctrl Pts',(-18.1935300219413,21.2578651462738,
-2.54181669139144));
#110695=CARTESIAN_POINT('Ctrl Pts',(-18.1851210863471,21.2556262877114,
-2.5423507562694));
#110696=CARTESIAN_POINT('Ctrl Pts',(-18.1255706058161,21.2393772875416,
-2.546158444936));
#110697=CARTESIAN_POINT('Ctrl Pts',(-18.0749617936444,21.2235030114371,
-2.54952798919886));
#110698=CARTESIAN_POINT('Ctrl Pts',(-18.0111276306136,21.2008144417576,
-2.5539054423609));
#110699=CARTESIAN_POINT('Ctrl Pts',(-17.9973002836321,21.1957366294717,
-2.55486148011119));
#110700=CARTESIAN_POINT('Ctrl Pts',(-17.8512118666701,21.1403516647053,
-2.56503816308134));
#110701=CARTESIAN_POINT('Ctrl Pts',(-17.7242571773421,21.0770481513458,
-2.57451403715176));
#110702=CARTESIAN_POINT('Ctrl Pts',(-17.5184240315459,20.947213134106,-2.59030455015483));
#110703=CARTESIAN_POINT('Ctrl Pts',(-17.436309447735,20.8867283503483,-2.59674775968453));
#110704=CARTESIAN_POINT('Ctrl Pts',(-17.3476241084051,20.8109591311117,
-2.60386081414444));
#110705=CARTESIAN_POINT('Ctrl Pts',(-17.3364903823184,20.8012434467342,
-2.60475701407788));
#110706=CARTESIAN_POINT('Ctrl Pts',(-17.3196643931974,20.7862472953726,
-2.60611660249239));
#110707=CARTESIAN_POINT('Ctrl Pts',(-17.3138981102644,20.7810509149454,
-2.60658348410878));
#110708=CARTESIAN_POINT('Ctrl Pts',(-17.3034585791741,20.7715385949314,
-2.60743053660901));
#110709=CARTESIAN_POINT('Ctrl Pts',(-17.2987759757018,20.7672331009249,
-2.60781114198737));
#110710=CARTESIAN_POINT('Ctrl Pts',(-17.2887079573,20.7578918097761,-2.6086309565558));
#110711=CARTESIAN_POINT('Ctrl Pts',(-17.2833292879657,20.7528488405803,
-2.6090698525835));
#110712=CARTESIAN_POINT('Ctrl Pts',(-17.2688147117739,20.7390969786577,
-2.61025683612894));
#110713=CARTESIAN_POINT('Ctrl Pts',(-17.2597300738474,20.7303342292723,
-2.61100259169567));
#110714=CARTESIAN_POINT('Ctrl Pts',(-17.2159005711963,20.687294411445,-2.61461529195019));
#110715=CARTESIAN_POINT('Ctrl Pts',(-17.1822681823724,20.6519024848284,
-2.61743270890948));
#110716=CARTESIAN_POINT('Ctrl Pts',(-17.1228450128653,20.5848742069277,
-2.62252290474575));
#110717=CARTESIAN_POINT('Ctrl Pts',(-17.0966885348781,20.5535953000447,
-2.62480790441187));
#110718=CARTESIAN_POINT('Ctrl Pts',(-16.9982908584207,20.4287718803747,
-2.63362798769001));
#110719=CARTESIAN_POINT('Ctrl Pts',(-16.9330313665142,20.3300026580496,
-2.63996611823286));
#110720=CARTESIAN_POINT('Ctrl Pts',(-16.8405335120332,20.1607642243681,
-2.65050122314283));
#110721=CARTESIAN_POINT('Ctrl Pts',(-16.8082092125215,20.0933806145278,
-2.65462412557213));
#110722=CARTESIAN_POINT('Ctrl Pts',(-16.7662502876465,19.992563733114,-2.66088047095741));
#110723=CARTESIAN_POINT('Ctrl Pts',(-16.7537678437019,19.9603738034231,
-2.66289083546881));
#110724=CARTESIAN_POINT('Ctrl Pts',(-16.7395821471637,19.9209582965944,
-2.66538429801141));
#110725=CARTESIAN_POINT('Ctrl Pts',(-16.7371218198147,19.9140084526406,
-2.66582513861859));
#110726=CARTESIAN_POINT('Ctrl Pts',(-16.7333370748242,19.903137262388,-2.66651677467955));
#110727=CARTESIAN_POINT('Ctrl Pts',(-16.7319877429683,19.8992245652255,
-2.66676611901149));
#110728=CARTESIAN_POINT('Ctrl Pts',(-16.7294965245968,19.8919313832965,
-2.66723170652321));
#110729=CARTESIAN_POINT('Ctrl Pts',(-16.7283517075889,19.8885519597664,
-2.66744777358066));
#110730=CARTESIAN_POINT('Ctrl Pts',(-16.7257699983805,19.8808670482946,
-2.66793985637005));
#110731=CARTESIAN_POINT('Ctrl Pts',(-16.7243384123481,19.8765598425575,
-2.66821617937816));
#110732=CARTESIAN_POINT('Ctrl Pts',(-16.7201155968612,19.8637168315464,
-2.66904158958636));
#110733=CARTESIAN_POINT('Ctrl Pts',(-16.717364860644,19.8551679591185,-2.66959296725551));
#110734=CARTESIAN_POINT('Ctrl Pts',(-16.696514408469,19.7889252941818,-2.67387905300726));
#110735=CARTESIAN_POINT('Ctrl Pts',(-16.6808412807037,19.7305026619888,
-2.67773826526523));
#110736=CARTESIAN_POINT('Ctrl Pts',(-16.6546081667227,19.6127910079383,
-2.68556636106876));
#110737=CARTESIAN_POINT('Ctrl Pts',(-16.6440334074358,19.5535573679836,
-2.6895310614893));
#110738=CARTESIAN_POINT('Ctrl Pts',(-16.6214478066949,19.3860943694899,
-2.70069458271644));
#110739=CARTESIAN_POINT('Ctrl Pts',(-16.6152391521043,19.2772627845727,
-2.70788802040985));
#110740=CARTESIAN_POINT('Ctrl Pts',(-16.618932834134,19.0936120799526,-2.71968874840913));
#110741=CARTESIAN_POINT('Ctrl Pts',(-16.6244037210298,19.0189200440966,
-2.72439646824398));
#110742=CARTESIAN_POINT('Ctrl Pts',(-16.6361827690023,18.9260358429179,
-2.73013199751174));
#110743=CARTESIAN_POINT('Ctrl Pts',(-16.6387933533262,18.9074364170283,
-2.73127465688877));
#110744=CARTESIAN_POINT('Ctrl Pts',(-16.6429520445461,18.8804239284348,
-2.73292609791404));
#110745=CARTESIAN_POINT('Ctrl Pts',(-16.6443041138119,18.8719820097731,
-2.73344105439541));
#110746=CARTESIAN_POINT('Ctrl Pts',(-16.6467656475359,18.8571874221772,
-2.73434156999406));
#110747=CARTESIAN_POINT('Ctrl Pts',(-16.6478530610269,18.8508312440371,
-2.73472782333231));
#110748=CARTESIAN_POINT('Ctrl Pts',(-16.6500219849041,18.8384928358023,
-2.73547640945912));
#110749=CARTESIAN_POINT('Ctrl Pts',(-16.6511002528523,18.8325101067406,
-2.73583884114541));
#110750=CARTESIAN_POINT('Ctrl Pts',(-16.6537412444267,18.818209811902,-2.73670387790195));
#110751=CARTESIAN_POINT('Ctrl Pts',(-16.6553281108973,18.8098967681258,
-2.73720571071442));
#110752=CARTESIAN_POINT('Ctrl Pts',(-16.6612450510339,18.7798784634625,
-2.73901427966966));
#110753=CARTESIAN_POINT('Ctrl Pts',(-16.6658656847988,18.7582314426846,
-2.74031175806969));
#110754=CARTESIAN_POINT('Ctrl Pts',(-16.712353133391,18.5560309379826,-2.75237824688537));
#110755=CARTESIAN_POINT('Ctrl Pts',(-16.7774183885294,18.3816418388984,
-2.76229334120737));
#110756=CARTESIAN_POINT('Ctrl Pts',(-16.9020359879003,18.1470238467712,
-2.77677482499561));
#110757=CARTESIAN_POINT('Ctrl Pts',(-16.9437063932024,18.0783110831566,
-2.78119041845442));
#110758=CARTESIAN_POINT('Ctrl Pts',(-17.0096028490715,17.9824053791749,
-2.78784616610286));
#110759=CARTESIAN_POINT('Ctrl Pts',(-17.0307864442922,17.9532029136862,
-2.78994434140374));
#110760=CARTESIAN_POINT('Ctrl Pts',(-17.0572428022676,17.918626182698,-2.79253527072107));
#110761=CARTESIAN_POINT('Ctrl Pts',(-17.0618127004352,17.9127186687016,
-2.79298179893197));
#110762=CARTESIAN_POINT('Ctrl Pts',(-17.0689763612735,17.9035587633895,
-2.79368041678069));
#110763=CARTESIAN_POINT('Ctrl Pts',(-17.0715486642688,17.9002895589227,
-2.79393100715533));
#110764=CARTESIAN_POINT('Ctrl Pts',(-17.0763437996697,17.894232124939,-2.79439769351204));
#110765=CARTESIAN_POINT('Ctrl Pts',(-17.0785640470679,17.8914419223009,
-2.79461360570287));
#110766=CARTESIAN_POINT('Ctrl Pts',(-17.083608277057,17.8851355654001,-2.79510374466763));
#110767=CARTESIAN_POINT('Ctrl Pts',(-17.0864364378377,17.8816228353622,
-2.79537826870676));
#110768=CARTESIAN_POINT('Ctrl Pts',(-17.0937670488373,17.8725771400632,
-2.79608904794247));
#110769=CARTESIAN_POINT('Ctrl Pts',(-17.0982862375867,17.8670578992284,
-2.79652646891331));
#110770=CARTESIAN_POINT('Ctrl Pts',(-17.1261971632411,17.8333198793415,
-2.79922281403875));
#110771=CARTESIAN_POINT('Ctrl Pts',(-17.1502891175498,17.8056915127307,
-2.8015278937844));
#110772=CARTESIAN_POINT('Ctrl Pts',(-17.2905032389765,17.6530819535127,
-2.81475349719218));
#110773=CARTESIAN_POINT('Ctrl Pts',(-17.4206816316658,17.5418716299619,
-2.82626472652731));
#110774=CARTESIAN_POINT('Ctrl Pts',(-17.6422116312476,17.3947469555842,
-2.84354642740194));
#110775=CARTESIAN_POINT('Ctrl Pts',(-17.7251041819546,17.347425360615,-2.84960310779911));
#110776=CARTESIAN_POINT('Ctrl Pts',(-17.8301604086857,17.2965234873061,
-2.85677377162878));
#110777=CARTESIAN_POINT('Ctrl Pts',(-17.8495462573935,17.287490718936,-2.85807727258134));
#110778=CARTESIAN_POINT('Ctrl Pts',(-17.8772887319129,17.275072325732,-2.85991548089011));
#110779=CARTESIAN_POINT('Ctrl Pts',(-17.8855347495824,17.2714441540344,
-2.86045849109549));
#110780=CARTESIAN_POINT('Ctrl Pts',(-17.8997939338557,17.265278583708,-2.86139175846869));
#110781=CARTESIAN_POINT('Ctrl Pts',(-17.9057960871884,17.2627161729118,
-2.86178286616702));
#110782=CARTESIAN_POINT('Ctrl Pts',(-17.9173067341061,17.2578649074406,
-2.86252963660411));
#110783=CARTESIAN_POINT('Ctrl Pts',(-17.9228132311356,17.2555715028454,
-2.86288545118564));
#110784=CARTESIAN_POINT('Ctrl Pts',(-17.937147622393,17.2496723324459,-2.86380803801545));
#110785=CARTESIAN_POINT('Ctrl Pts',(-17.9459903797506,17.2461028591481,
-2.86437357822826));
#110786=CARTESIAN_POINT('Ctrl Pts',(-17.9761758811916,17.2341547088343,
-2.86629213933818));
#110787=CARTESIAN_POINT('Ctrl Pts',(-17.997630959482,17.226062873325,-2.86763553056476));
#110788=CARTESIAN_POINT('Ctrl Pts',(-18.1851804446528,17.1587877317944,
-2.87921439783776));
#110789=CARTESIAN_POINT('Ctrl Pts',(-18.3579315083373,17.120220899497,-2.88869057347339));
#110790=CARTESIAN_POINT('Ctrl Pts',(-18.6195061113945,17.0953327563968,
-2.90298930981596));
#110791=CARTESIAN_POINT('Ctrl Pts',(-18.7059476050395,17.0924232517146,
-2.90772198839001));
#110792=CARTESIAN_POINT('Ctrl Pts',(-18.8299768237063,17.0958411945691,
-2.91480714904523));
#110793=CARTESIAN_POINT('Ctrl Pts',(-18.8675994300068,17.0978840258145,
-2.91699576751067));
#110794=CARTESIAN_POINT('Ctrl Pts',(-18.9126832038257,17.1015407057472,
-2.91968698980269));
#110795=CARTESIAN_POINT('Ctrl Pts',(-18.9202181521132,17.1021925177128,
-2.92013908719328));
#110796=CARTESIAN_POINT('Ctrl Pts',(-18.9319121858262,17.1032672744012,
-2.92084453786562));
#110797=CARTESIAN_POINT('Ctrl Pts',(-18.9360738713595,17.1036621946923,
-2.92109634407894));
#110798=CARTESIAN_POINT('Ctrl Pts',(-18.9437813106418,17.104416627949,-2.92156412314885));
#110799=CARTESIAN_POINT('Ctrl Pts',(-18.9473273364876,17.1047727689968,
-2.92177990479591));
#110800=CARTESIAN_POINT('Ctrl Pts',(-18.9553313930585,17.1055970676607,
-2.92226824039758));
#110801=CARTESIAN_POINT('Ctrl Pts',(-18.9597888206167,17.1060704285688,
-2.92254108223638));
#110802=CARTESIAN_POINT('Ctrl Pts',(-18.9729099210101,17.1075059935572,
-2.92334678585299));
#110803=CARTESIAN_POINT('Ctrl Pts',(-18.9815690702414,17.1085075422358,
-2.923881782501));
#110804=CARTESIAN_POINT('Ctrl Pts',(-19.0431294769498,17.1160134075918,
-2.92770739209667));
#110805=CARTESIAN_POINT('Ctrl Pts',(-19.0957702381481,17.1244595338442,
-2.93109490621968));
#110806=CARTESIAN_POINT('Ctrl Pts',(-19.1656348808281,17.1383923317878,
-2.93569896422243));
#110807=CARTESIAN_POINT('Ctrl Pts',(-19.183192927769,17.1421266581325,-2.93686531945922));
#110808=CARTESIAN_POINT('Ctrl Pts',(-19.24774156537,17.156715585646,-2.94118294851364));
#110809=CARTESIAN_POINT('Ctrl Pts',(-19.2944039419844,17.1689515089548,
-2.94436226767155));
#110810=CARTESIAN_POINT('Ctrl Pts',(-19.4453996142591,17.2141115457453,
-2.95477317648947));
#110811=CARTESIAN_POINT('Ctrl Pts',(-19.5476143332185,17.2535301809381,
-2.96200574809195));
#110812=CARTESIAN_POINT('Ctrl Pts',(-19.714619340497,17.3332881506789,-2.97390173133479));
#110813=CARTESIAN_POINT('Ctrl Pts',(-19.7811165193729,17.3695426221303,
-2.97866453071452));
#110814=CARTESIAN_POINT('Ctrl Pts',(-19.8616162957819,17.4192055102461,
-2.98445948256182));
#110815=CARTESIAN_POINT('Ctrl Pts',(-19.8775637363913,17.4293412164024,
-2.98560917885865));
#110816=CARTESIAN_POINT('Ctrl Pts',(-19.9005445937735,17.4443828482994,
-2.98726884991084));
#110817=CARTESIAN_POINT('Ctrl Pts',(-19.9076869402443,17.4491199190584,
-2.98778508636765));
#110818=CARTESIAN_POINT('Ctrl Pts',(-19.9201552702724,17.4574988454538,
-2.98868707888915));
#110819=CARTESIAN_POINT('Ctrl Pts',(-19.9254937013597,17.4611218941769,
-2.98907353619654));
#110820=CARTESIAN_POINT('Ctrl Pts',(-19.9358248196863,17.4682025411038,
-2.98982196596707));
#110821=CARTESIAN_POINT('Ctrl Pts',(-19.9408193501042,17.4716573260724,
-2.99018403992115));
#110822=CARTESIAN_POINT('Ctrl Pts',(-19.9527191944609,17.4799645432514,
-2.99104734627265));
#110823=CARTESIAN_POINT('Ctrl Pts',(-19.9596105273439,17.4848368947673,
-2.99154781349463));
#110824=CARTESIAN_POINT('Ctrl Pts',(-19.984347160739,17.5025491562118,-2.99334630862947));
#110825=CARTESIAN_POINT('Ctrl Pts',(-20.0020217238731,17.5156259205698,
-2.99463521496988));
#110826=CARTESIAN_POINT('Ctrl Pts',(-20.16790647912,17.6424036452805,-3.00677958094477));
#110827=CARTESIAN_POINT('Ctrl Pts',(-20.3006546993801,17.7749703104854,
-3.01676512932791));
#110828=CARTESIAN_POINT('Ctrl Pts',(-20.4625579748485,17.9862256044517,
-3.03127850219662));
#110829=CARTESIAN_POINT('Ctrl Pts',(-20.5072417077249,18.0518637374812,
-3.03564442815817));
#110830=CARTESIAN_POINT('Ctrl Pts',(-20.5665927235223,18.1505398963798,
-3.0422326101284));
#110831=CARTESIAN_POINT('Ctrl Pts',(-20.5842696290703,18.1816926219035,
-3.04431618330247));
#110832=CARTESIAN_POINT('Ctrl Pts',(-20.6046593321897,18.2198500553934,
-3.04689091169714));
#110833=CARTESIAN_POINT('Ctrl Pts',(-20.6081371493158,18.2264419815935,
-3.0473365138029));
#110834=CARTESIAN_POINT('Ctrl Pts',(-20.6135001086041,18.2367384242285,
-3.04803399505739));
#110835=CARTESIAN_POINT('Ctrl Pts',(-20.6154093111171,18.2404304354519,
-3.04828438282849));
#110836=CARTESIAN_POINT('Ctrl Pts',(-20.6189363568608,18.2473005404384,
-3.04875088902753));
#110837=CARTESIAN_POINT('Ctrl Pts',(-20.6205570469706,18.2504771081894,
-3.04896682490641));
#110838=CARTESIAN_POINT('Ctrl Pts',(-20.6242112018844,18.2576842116327,
-3.04945727315536));
#110839=CARTESIAN_POINT('Ctrl Pts',(-20.6262397950634,18.2617171458489,
-3.04973208439025));
#110840=CARTESIAN_POINT('Ctrl Pts',(-20.6322139852811,18.2736893438273,
-3.05054890868033));
#110841=CARTESIAN_POINT('Ctrl Pts',(-20.6361225689186,18.2816468235407,
-3.05109314375318));
#110842=CARTESIAN_POINT('Ctrl Pts',(-20.6648569174112,18.3410876886567,
-3.05516698365295));
#110843=CARTESIAN_POINT('Ctrl Pts',(-20.6876363765022,18.39352857509,-3.05880793160253));
#110844=CARTESIAN_POINT('Ctrl Pts',(-20.7131595094723,18.459467874377,-3.06338857213167));
#110845=CARTESIAN_POINT('Ctrl Pts',(-20.7179317366394,18.4721579512576,
-3.06427026063966));
#110846=CARTESIAN_POINT('Ctrl Pts',(-20.7225805974208,18.4848896725968,
-3.06515445288237));
#110847=CARTESIAN_POINT('',(-20.8479141186681,19.210171541465,-2.08900434294145));
#110848=CARTESIAN_POINT('Ctrl Pts',(-20.7202231698227,18.4857291668958,
-2.84456322999407));
#110849=CARTESIAN_POINT('Ctrl Pts',(-20.6328470740777,18.2413750955877,
-2.82899806899323));
#110850=CARTESIAN_POINT('Ctrl Pts',(-20.1480309870729,17.3916716763849,
-2.77104097243191));
#110851=CARTESIAN_POINT('Ctrl Pts',(-18.3741968228298,16.7337288824509,
-2.6706919403101));
#110852=CARTESIAN_POINT('Ctrl Pts',(-16.4562523864159,18.1726376448454,
-2.54351613362869));
#110853=CARTESIAN_POINT('Ctrl Pts',(-16.6280000106062,20.564179464316,-2.41634032694724));
#110854=CARTESIAN_POINT('Ctrl Pts',(-18.731871915622,21.7142630277803,-2.28916452026582));
#110855=CARTESIAN_POINT('Ctrl Pts',(-20.5383022256027,20.7307617397078,
-2.18006983762423));
#110856=CARTESIAN_POINT('Ctrl Pts',(-20.8463944855641,19.6158003448226,
-2.11336709054312));
#110857=CARTESIAN_POINT('Ctrl Pts',(-20.8478239987731,19.2101685861784,
-2.0890562790225));
#110858=CARTESIAN_POINT('Ctrl Pts',(-20.8509998750783,19.2102727321581,
-2.08722602201616));
#110859=CARTESIAN_POINT('Ctrl Pts',(-20.850932996752,19.0155969878683,-2.07601666321716));
#110860=CARTESIAN_POINT('Ctrl Pts',(-20.8240164305583,18.8218628606765,
-2.06573534679094));
#110861=CARTESIAN_POINT('Ctrl Pts',(-20.7567162189418,18.584055871884,-2.05215244185046));
#110862=CARTESIAN_POINT('Ctrl Pts',(-20.7405653205142,18.5341439975041,
-2.04923747298217));
#110863=CARTESIAN_POINT('Ctrl Pts',(-20.7225806143688,18.484889719012,-2.04625075898636));
#110864=CARTESIAN_POINT('Origin',(-18.734,19.211,0.));
#110865=CARTESIAN_POINT('',(-20.7225806756344,18.4848898867987,-1.24458630806144));
#110866=CARTESIAN_POINT('',(-20.7225806136401,18.4848897170162,-1.46829797183507));
#110867=CARTESIAN_POINT('',(-20.7225806137986,18.4848897174502,0.));
#110868=CARTESIAN_POINT('Ctrl Pts',(-20.7225806136401,18.4848897170162,
-1.46829797183507));
#110869=CARTESIAN_POINT('Ctrl Pts',(-20.772093170878,18.6204885561492,-1.4767475415403));
#110870=CARTESIAN_POINT('Ctrl Pts',(-20.8076106590459,18.7608045197434,
-1.48469153836204));
#110871=CARTESIAN_POINT('Ctrl Pts',(-20.8435716232105,19.0058873147326,
-1.49816093193042));
#110872=CARTESIAN_POINT('Ctrl Pts',(-20.8510665768484,19.1090662014719,
-1.5037241301894));
#110873=CARTESIAN_POINT('Ctrl Pts',(-20.8509605930383,19.2724280292508,
-1.5128625274986));
#110874=CARTESIAN_POINT('Ctrl Pts',(-20.848366219973,19.3324481090795,-1.51629225644068));
#110875=CARTESIAN_POINT('Ctrl Pts',(-20.8424571662823,19.4012045864611,
-1.52038549800654));
#110876=CARTESIAN_POINT('Ctrl Pts',(-20.84163261838,19.4101334885926,-1.52092026133344));
#110877=CARTESIAN_POINT('Ctrl Pts',(-20.8403055953013,19.423570727867,-1.52173022272583));
#110878=CARTESIAN_POINT('Ctrl Pts',(-20.8398453012565,19.4280832592346,
-1.52200310844775));
#110879=CARTESIAN_POINT('Ctrl Pts',(-20.8389970518347,19.4361424913529,
-1.52249210538345));
#110880=CARTESIAN_POINT('Ctrl Pts',(-20.8386146299038,19.4396897220715,
-1.52270790270283));
#110881=CARTESIAN_POINT('Ctrl Pts',(-20.837768977974,19.4473519291442,-1.5231752774535));
#110882=CARTESIAN_POINT('Ctrl Pts',(-20.8373026477048,19.4514664603963,
-1.52342702188824));
#110883=CARTESIAN_POINT('Ctrl Pts',(-20.8359714187376,19.4629119818602,
-1.52412939672326));
#110884=CARTESIAN_POINT('Ctrl Pts',(-20.8350802526499,19.4702397732347,
-1.5245814667027));
#110885=CARTESIAN_POINT('Ctrl Pts',(-20.8297855229006,19.5119550389898,
-1.5271680133266));
#110886=CARTESIAN_POINT('Ctrl Pts',(-20.8245763666059,19.5462327957154,
-1.52934381699349));
#110887=CARTESIAN_POINT('Ctrl Pts',(-20.8054071890936,19.6544149896487,
-1.53633891098771));
#110888=CARTESIAN_POINT('Ctrl Pts',(-20.7883503424776,19.7277085403984,
-1.54126752850267));
#110889=CARTESIAN_POINT('Ctrl Pts',(-20.7136651524747,19.9855767263582,
-1.55897626805703));
#110890=CARTESIAN_POINT('Ctrl Pts',(-20.6347144920359,20.1630288020327,
-1.57174491669585));
#110891=CARTESIAN_POINT('Ctrl Pts',(-20.52155967755,20.3453590042295,-1.58493000273531));
#110892=CARTESIAN_POINT('Ctrl Pts',(-20.5100907630276,20.3632333115886,
-1.58622485581085));
#110893=CARTESIAN_POINT('Ctrl Pts',(-20.4937578174105,20.3878647368295,
-1.58801298157456));
#110894=CARTESIAN_POINT('Ctrl Pts',(-20.4891202632915,20.3947698463815,
-1.58851468253942));
#110895=CARTESIAN_POINT('Ctrl Pts',(-20.4810444645849,20.4066425607041,
-1.58937810281685));
#110896=CARTESIAN_POINT('Ctrl Pts',(-20.4776254564377,20.4116230728427,
-1.58974054362169));
#110897=CARTESIAN_POINT('Ctrl Pts',(-20.4705005819946,20.4219073417681,
-1.59048948289309));
#110898=CARTESIAN_POINT('Ctrl Pts',(-20.4667916223787,20.4272088868545,
-1.59087585834058));
#110899=CARTESIAN_POINT('Ctrl Pts',(-20.4580472064134,20.4395868545563,
-1.5917787065444));
#110900=CARTESIAN_POINT('Ctrl Pts',(-20.4529923688728,20.4466494924997,
-1.59229442933029));
#110901=CARTESIAN_POINT('Ctrl Pts',(-20.4364321481621,20.4694891976478,
-1.59396426284884));
#110902=CARTESIAN_POINT('Ctrl Pts',(-20.4247517069832,20.4851385257338,
-1.59511159306344));
#110903=CARTESIAN_POINT('Ctrl Pts',(-20.3638544262758,20.5644156951665,
-1.6009440405323));
#110904=CARTESIAN_POINT('Ctrl Pts',(-20.3112538404237,20.6253662372658,
-1.60549253391176));
#110905=CARTESIAN_POINT('Ctrl Pts',(-20.1384830030225,20.8039024264036,
-1.61926738115335));
#110906=CARTESIAN_POINT('Ctrl Pts',(-20.0077164891844,20.9102791333806,
-1.62810924859928));
#110907=CARTESIAN_POINT('Ctrl Pts',(-19.8645527343082,21.0008440070415,
-1.63762177446481));
#110908=CARTESIAN_POINT('Ctrl Pts',(-19.8633406036649,21.001609073889,-1.63770230688805));
#110909=CARTESIAN_POINT('Ctrl Pts',(-19.8165544504403,21.0310729309989,
-1.64081045970006));
#110910=CARTESIAN_POINT('Ctrl Pts',(-19.7699065971989,21.0580208684212,
-1.64389973656495));
#110911=CARTESIAN_POINT('Ctrl Pts',(-19.7145584032438,21.087238414556,-1.64761367364294));
#110912=CARTESIAN_POINT('Ctrl Pts',(-19.7068050584584,21.0912701089764,
-1.64813501313869));
#110913=CARTESIAN_POINT('Ctrl Pts',(-19.6950331591432,21.0972991287085,
-1.64892852740314));
#110914=CARTESIAN_POINT('Ctrl Pts',(-19.6910327410687,21.0993319272865,
-1.649198526796));
#110915=CARTESIAN_POINT('Ctrl Pts',(-19.683843252723,21.1029565268024,-1.64968443062165));
#110916=CARTESIAN_POINT('Ctrl Pts',(-19.6806566008649,21.1045530052785,
-1.6499000375978));
#110917=CARTESIAN_POINT('Ctrl Pts',(-19.6737268085872,21.108002891657,-1.65036942735312));
#110918=CARTESIAN_POINT('Ctrl Pts',(-19.6699822597049,21.1098532472402,
-1.65062339025646));
#110919=CARTESIAN_POINT('Ctrl Pts',(-19.6594568308272,21.1150156524095,
-1.65133810705894));
#110920=CARTESIAN_POINT('Ctrl Pts',(-19.6526637603123,21.1183025040342,
-1.6518003822164));
#110921=CARTESIAN_POINT('Ctrl Pts',(-19.6121136771161,21.1376559227571,
-1.65456514608512));
#110922=CARTESIAN_POINT('Ctrl Pts',(-19.577955653816,21.1528612546117,-1.65691576629389));
#110923=CARTESIAN_POINT('Ctrl Pts',(-19.4646081386315,21.1997621018972,
-1.66474457719752));
#110924=CARTESIAN_POINT('Ctrl Pts',(-19.3839070776935,21.2275767701418,
-1.67036055457777));
#110925=CARTESIAN_POINT('Ctrl Pts',(-19.1303549397287,21.2981622714081,
-1.68774770695599));
#110926=CARTESIAN_POINT('Ctrl Pts',(-18.9535869921731,21.3240900494598,
-1.69943901710199));
#110927=CARTESIAN_POINT('Ctrl Pts',(-18.7528396253182,21.3280389508183,
-1.71179546537254));
#110928=CARTESIAN_POINT('Ctrl Pts',(-18.7300373791083,21.3281190831423,
-1.71318717086491));
#110929=CARTESIAN_POINT('Ctrl Pts',(-18.6977235695387,21.3277105496945,
-1.71514332857322));
#110930=CARTESIAN_POINT('Ctrl Pts',(-18.6882103733659,21.3275261267726,
-1.71571725069181));
#110931=CARTESIAN_POINT('Ctrl Pts',(-18.6727395335275,21.3271218514576,
-1.71664746726135));
#110932=CARTESIAN_POINT('Ctrl Pts',(-18.666781083937,21.3269409617051,-1.71700497755867));
#110933=CARTESIAN_POINT('Ctrl Pts',(-18.6542978150237,21.3265092049677,
-1.71775243060923));
#110934=CARTESIAN_POINT('Ctrl Pts',(-18.6477732235398,21.3262533132198,
-1.71814221190239));
#110935=CARTESIAN_POINT('Ctrl Pts',(-18.6322313311064,21.3255717363993,
-1.71906862383351));
#110936=CARTESIAN_POINT('Ctrl Pts',(-18.6232153165642,21.3251185511004,
-1.7196043871257));
#110937=CARTESIAN_POINT('Ctrl Pts',(-18.5927419619009,21.3233913451983,
-1.72140982004915));
#110938=CARTESIAN_POINT('Ctrl Pts',(-18.5713007730654,21.321848180288,-1.72267105502257));
#110939=CARTESIAN_POINT('Ctrl Pts',(-18.37109355362,21.3043700943778,-1.73437218530679));
#110940=CARTESIAN_POINT('Ctrl Pts',(-18.1950140076912,21.2660913668851,
-1.74401510710511));
#110941=CARTESIAN_POINT('Ctrl Pts',(-17.9123263109276,21.1657520524479,
-1.76034028089886));
#110942=CARTESIAN_POINT('Ctrl Pts',(-17.8024542251927,21.1158404754064,
-1.76694993789784));
#110943=CARTESIAN_POINT('Ctrl Pts',(-17.6891590166171,21.0522187560071,
-1.77465079425141));
#110944=CARTESIAN_POINT('Ctrl Pts',(-17.680910115097,21.0475132383796,-1.77521686369375));
#110945=CARTESIAN_POINT('Ctrl Pts',(-17.6687297401433,21.0404560003738,
-1.77606114966729));
#110946=CARTESIAN_POINT('Ctrl Pts',(-17.664773660047,21.0381466872926,-1.7763366940007));
#110947=CARTESIAN_POINT('Ctrl Pts',(-17.6577462647211,21.0340138933654,
-1.77682858204549));
#110948=CARTESIAN_POINT('Ctrl Pts',(-17.6546720386063,21.0321954616757,
-1.7770445967854));
#110949=CARTESIAN_POINT('Ctrl Pts',(-17.6480700897573,21.0282677632469,
-1.77751029947401));
#110950=CARTESIAN_POINT('Ctrl Pts',(-17.6445439550583,21.0261560315225,
-1.77776014303231));
#110951=CARTESIAN_POINT('Ctrl Pts',(-17.6348221353206,21.0202952947674,
-1.77845200097139));
#110952=CARTESIAN_POINT('Ctrl Pts',(-17.6286395709653,21.0165247880609,
-1.77889538694874));
#110953=CARTESIAN_POINT('Ctrl Pts',(-17.5947837336046,20.9956383573915,
-1.78134158865437));
#110954=CARTESIAN_POINT('Ctrl Pts',(-17.5674901691052,20.9779188757617,
-1.78338075026793));
#110955=CARTESIAN_POINT('Ctrl Pts',(-17.4062312191767,20.8678617196679,
-1.79578677801862));
#110956=CARTESIAN_POINT('Ctrl Pts',(-17.2828694487212,20.760961530764,-1.80674351524227));
#110957=CARTESIAN_POINT('Ctrl Pts',(-17.0940656621517,20.5548559903665,
-1.82500098322813));
#110958=CARTESIAN_POINT('Ctrl Pts',(-17.0224172982632,20.4623296992898,
-1.8324417104591));
#110959=CARTESIAN_POINT('Ctrl Pts',(-16.9509757770334,20.3523666389927,
-1.84044866088052));
#110960=CARTESIAN_POINT('Ctrl Pts',(-16.9433122852977,20.3403054097198,
-1.84131663452484));
#110961=CARTESIAN_POINT('Ctrl Pts',(-16.9313098083461,20.3209858338611,
-1.84269093951051));
#110962=CARTESIAN_POINT('Ctrl Pts',(-16.9268912772551,20.3137776502433,
-1.84320019890914));
#110963=CARTESIAN_POINT('Ctrl Pts',(-16.9191746638351,20.3010182054698,
-1.84409557502407));
#110964=CARTESIAN_POINT('Ctrl Pts',(-16.9158585973788,20.2954779991077,
-1.84448234786525));
#110965=CARTESIAN_POINT('Ctrl Pts',(-16.9090523326695,20.2839876954241,
-1.84528041501967));
#110966=CARTESIAN_POINT('Ctrl Pts',(-16.9055657621033,20.2780355300763,
-1.84569157395204));
#110967=CARTESIAN_POINT('Ctrl Pts',(-16.8966908943633,20.262713400558,-1.8467442818472));
#110968=CARTESIAN_POINT('Ctrl Pts',(-16.8913451090216,20.2533189463313,
-1.84738428951001));
#110969=CARTESIAN_POINT('Ctrl Pts',(-16.8693339854494,20.2139389280165,
-1.8500449507682));
#110970=CARTESIAN_POINT('Ctrl Pts',(-16.853326234936,20.1835904714479,-1.85204207564392));
#110971=CARTESIAN_POINT('Ctrl Pts',(-16.8135459453665,20.1035143011146,
-1.85718614484259));
#110972=CARTESIAN_POINT('Ctrl Pts',(-16.790964549502,20.0532229141713,-1.86029370021906));
#110973=CARTESIAN_POINT('Ctrl Pts',(-16.7295083369658,19.9006802098619,
-1.86943810277065));
#110974=CARTESIAN_POINT('Ctrl Pts',(-16.6965650202614,19.7962394433127,
-1.87532622032092));
#110975=CARTESIAN_POINT('Ctrl Pts',(-16.6614979198788,19.6451828366451,
-1.88376907075576));
#110976=CARTESIAN_POINT('Ctrl Pts',(-16.6526043735314,19.6003219961865,
-1.88626911846589));
#110977=CARTESIAN_POINT('Ctrl Pts',(-16.6414625464269,19.5327080713401,
-1.89006889938615));
#110978=CARTESIAN_POINT('Ctrl Pts',(-16.6381185040672,19.5101484261164,
-1.89134199193598));
#110979=CARTESIAN_POINT('Ctrl Pts',(-16.6349997254098,19.4864777571354,
-1.89268722023571));
#110980=CARTESIAN_POINT('Ctrl Pts',(-16.6348606066572,19.4854156604791,
-1.89274760014244));
#110981=CARTESIAN_POINT('Ctrl Pts',(-16.6322661713896,19.4654911271904,
-1.89388068451132));
#110982=CARTESIAN_POINT('Ctrl Pts',(-16.6300644480917,19.4465970583556,
-1.89496155260961));
#110983=CARTESIAN_POINT('Ctrl Pts',(-16.6247547778914,19.3949922707455,
-1.89793716880863));
#110984=CARTESIAN_POINT('Ctrl Pts',(-16.6221534413677,19.3622362653008,
-1.89985157408718));
#110985=CARTESIAN_POINT('Ctrl Pts',(-16.6199303411559,19.3225610941034,
-1.90221548195122));
#110986=CARTESIAN_POINT('Ctrl Pts',(-16.6195787148595,19.3156853674982,
-1.90262678473982));
#110987=CARTESIAN_POINT('Ctrl Pts',(-16.6190558028044,19.3043793296246,
-1.90330597445504));
#110988=CARTESIAN_POINT('Ctrl Pts',(-16.618864881926,19.2999499180403,-1.90357278659488));
#110989=CARTESIAN_POINT('Ctrl Pts',(-16.6185457019116,19.2919616848831,
-1.9040553258584));
#110990=CARTESIAN_POINT('Ctrl Pts',(-16.6184125073555,19.2884031158922,
-1.90427077371997));
#110991=CARTESIAN_POINT('Ctrl Pts',(-16.6181411073559,19.2806272278032,
-1.9047426280809));
#110992=CARTESIAN_POINT('Ctrl Pts',(-16.6180065331723,19.276409877377,-1.904999230178));
#110993=CARTESIAN_POINT('Ctrl Pts',(-16.6176607291121,19.2644514682656,
-1.90572872268441));
#110994=CARTESIAN_POINT('Ctrl Pts',(-16.6174793676046,19.2567097074783,
-1.90620323481775));
#110995=CARTESIAN_POINT('Ctrl Pts',(-16.6166052469029,19.20797783466,-1.90920352792312));
#110996=CARTESIAN_POINT('Ctrl Pts',(-16.6170608681158,19.1669787141585,
-1.91178725615409));
#110997=CARTESIAN_POINT('Ctrl Pts',(-16.6260552817034,18.943087572951,-1.92613099367957));
#110998=CARTESIAN_POINT('Ctrl Pts',(-16.6571021423828,18.7618768183812,
-1.93851336704575));
#110999=CARTESIAN_POINT('Ctrl Pts',(-16.7370944515095,18.5025908417339,
-1.95601438523293));
#111000=CARTESIAN_POINT('Ctrl Pts',(-16.7683562975834,18.4199730547995,
-1.96157153686915));
#111001=CARTESIAN_POINT('Ctrl Pts',(-16.8103162345117,18.3270788052049,
-1.96779041290174));
#111002=CARTESIAN_POINT('Ctrl Pts',(-16.8160647347727,18.3146740323007,
-1.96862036383626));
#111003=CARTESIAN_POINT('Ctrl Pts',(-16.8254845392132,18.2948525254036,
-1.9699459384234));
#111004=CARTESIAN_POINT('Ctrl Pts',(-16.8290797910932,18.2874002706771,
-1.97044417575424));
#111005=CARTESIAN_POINT('Ctrl Pts',(-16.8355458639991,18.2741957411976,
-1.97132681299776));
#111006=CARTESIAN_POINT('Ctrl Pts',(-16.8383993534999,18.2684351395203,
-1.97171181019933));
#111007=CARTESIAN_POINT('Ctrl Pts',(-16.8444044030833,18.2564497613088,
-1.97251273631025));
#111008=CARTESIAN_POINT('Ctrl Pts',(-16.8475605890665,18.2502273792721,
-1.97292849744536));
#111009=CARTESIAN_POINT('Ctrl Pts',(-16.8558480976322,18.2340869402244,
-1.97400688831941));
#111010=CARTESIAN_POINT('Ctrl Pts',(-16.8610272763885,18.2241935962108,
-1.97466782663415));
#111011=CARTESIAN_POINT('Ctrl Pts',(-16.8839668193809,18.1812054106382,
-1.97753995334988));
#111012=CARTESIAN_POINT('Ctrl Pts',(-16.9025284906629,18.1485443389106,
-1.97972257113581));
#111013=CARTESIAN_POINT('Ctrl Pts',(-16.9542722721378,18.0628859284714,
-1.98546413999428));
#111014=CARTESIAN_POINT('Ctrl Pts',(-16.9889498675745,18.0108343342411,
-1.98897057598798));
#111015=CARTESIAN_POINT('Ctrl Pts',(-17.0946125412111,17.8665172824652,
-1.998860473838));
#111016=CARTESIAN_POINT('Ctrl Pts',(-17.1709627413942,17.778470936924,-2.00509548245638));
#111017=CARTESIAN_POINT('Ctrl Pts',(-17.3255285815601,17.6273782381556,
-2.01692457769316));
#111018=CARTESIAN_POINT('Ctrl Pts',(-17.4017323359465,17.5627563211379,
-2.02247378546111));
#111019=CARTESIAN_POINT('Ctrl Pts',(-17.4900147963413,17.4980248685897,
-2.02895931383772));
#111020=CARTESIAN_POINT('Ctrl Pts',(-17.4978721726306,17.4923461738664,
-2.02953703118549));
#111021=CARTESIAN_POINT('Ctrl Pts',(-17.5095306305389,17.484041661526,-2.03039538901899));
#111022=CARTESIAN_POINT('Ctrl Pts',(-17.5133018765579,17.4813739045473,
-2.03067322641621));
#111023=CARTESIAN_POINT('Ctrl Pts',(-17.5200076965833,17.4766631027844,
-2.03116763491802));
#111024=CARTESIAN_POINT('Ctrl Pts',(-17.5229387469449,17.4746151270706,
-2.03138386406435));
#111025=CARTESIAN_POINT('Ctrl Pts',(-17.5292296625561,17.4702432327415,
-2.03184824767471));
#111026=CARTESIAN_POINT('Ctrl Pts',(-17.5325910193304,17.4679216456925,
-2.03209654840715));
#111027=CARTESIAN_POINT('Ctrl Pts',(-17.541836086478,17.4615758043646,-2.03277989674342));
#111028=CARTESIAN_POINT('Ctrl Pts',(-17.5477333727836,17.4575715586888,
-2.03321626197525));
#111029=CARTESIAN_POINT('Ctrl Pts',(-17.5793230731723,17.4363545204237,
-2.03555571816893));
#111030=CARTESIAN_POINT('Ctrl Pts',(-17.6053686935918,17.4196774370775,
-2.03749158792104));
#111031=CARTESIAN_POINT('Ctrl Pts',(-17.6853024591858,17.3709309344064,
-2.04343173718327));
#111032=CARTESIAN_POINT('Ctrl Pts',(-17.7402568165067,17.340680753308,-2.04751346858103));
#111033=CARTESIAN_POINT('Ctrl Pts',(-17.9272150449388,17.2483353736808,
-2.06121640637012));
#111034=CARTESIAN_POINT('Ctrl Pts',(-18.0643009772396,17.1974296987275,
-2.07093960091191));
#111035=CARTESIAN_POINT('Ctrl Pts',(-18.2780045266389,17.1423391488082,
-2.08506738200193));
#111036=CARTESIAN_POINT('Ctrl Pts',(-18.3514180325007,17.1275118696366,
-2.08975426356528));
#111037=CARTESIAN_POINT('Ctrl Pts',(-18.438452373882,17.1146906740026,-2.09511762195096));
#111038=CARTESIAN_POINT('Ctrl Pts',(-18.451452095435,17.112898981609,-2.09591379190503));
#111039=CARTESIAN_POINT('Ctrl Pts',(-18.4726000748713,17.1101843723045,
-2.09720120544719));
#111040=CARTESIAN_POINT('Ctrl Pts',(-18.4807383632071,17.1091877418027,
-2.09769476491574));
#111041=CARTESIAN_POINT('Ctrl Pts',(-18.495239242451,17.1074973828996,-2.0985709262653));
#111042=CARTESIAN_POINT('Ctrl Pts',(-18.5015995392823,17.1067851852185,
-2.09895410615008));
#111043=CARTESIAN_POINT('Ctrl Pts',(-18.5150065447146,17.1053454580934,
-2.09975950511818));
#111044=CARTESIAN_POINT('Ctrl Pts',(-18.5220538836354,17.1046244330745,
-2.10018151485112));
#111045=CARTESIAN_POINT('Ctrl Pts',(-18.5407000552306,17.1028112387086,
-2.1012946051871));
#111046=CARTESIAN_POINT('Ctrl Pts',(-18.5523046151238,17.1017794052805,
-2.10198378334474));
#111047=CARTESIAN_POINT('Ctrl Pts',(-18.6062150455316,17.0974341198738,
-2.105169574526));
#111048=CARTESIAN_POINT('Ctrl Pts',(-18.6486076683341,17.0952972237828,
-2.10762913198384));
#111049=CARTESIAN_POINT('Ctrl Pts',(-18.7655036106586,17.0929244791949,
-2.11431062805601));
#111050=CARTESIAN_POINT('Ctrl Pts',(-18.8400009351297,17.0953437149919,
-2.1184545985267));
#111051=CARTESIAN_POINT('Ctrl Pts',(-19.0801363246528,17.1158609224158,
-2.13168202061258));
#111052=CARTESIAN_POINT('Ctrl Pts',(-19.2437801056489,17.1495610455256,
-2.14046030295509));
#111053=CARTESIAN_POINT('Ctrl Pts',(-19.4349847888982,17.2131174368166,
-2.15199060397981));
#111054=CARTESIAN_POINT('Ctrl Pts',(-19.4679224323766,17.2249808776535,
-2.15402679701654));
#111055=CARTESIAN_POINT('Ctrl Pts',(-19.5071002780485,17.2401995633245,
-2.15652622605923));
#111056=CARTESIAN_POINT('Ctrl Pts',(-19.5136391089855,17.2427771320967,
-2.15694601087442));
#111057=CARTESIAN_POINT('Ctrl Pts',(-19.5243224062948,17.2470500148479,
-2.15763636305506));
#111058=CARTESIAN_POINT('Ctrl Pts',(-19.5284746031473,17.2487260246904,
-2.15790579442479));
#111059=CARTESIAN_POINT('Ctrl Pts',(-19.535921727548,17.2517595241352,-2.15839109267274));
#111060=CARTESIAN_POINT('Ctrl Pts',(-19.5392185696694,17.2531121701846,
-2.15860666532094));
#111061=CARTESIAN_POINT('Ctrl Pts',(-19.5463789673075,17.2560711214286,
-2.15907646932416));
#111062=CARTESIAN_POINT('Ctrl Pts',(-19.5502411304838,17.257680537392,-2.15933088347273));
#111063=CARTESIAN_POINT('Ctrl Pts',(-19.5609462500667,17.2621787995516,
-2.1600388273396));
#111064=CARTESIAN_POINT('Ctrl Pts',(-19.5677787346432,17.2650921939319,
-2.16049380715666));
#111065=CARTESIAN_POINT('Ctrl Pts',(-19.607532075362,17.2822909572066,-2.16315874751795));
#111066=CARTESIAN_POINT('Ctrl Pts',(-19.6400986699825,17.2973747219567,
-2.16541301610423));
#111067=CARTESIAN_POINT('Ctrl Pts',(-19.7438174942051,17.3486549461156,
-2.17278807546737));
#111068=CARTESIAN_POINT('Ctrl Pts',(-19.8133083911187,17.3880485025383,
-2.17803105458147));
#111069=CARTESIAN_POINT('Ctrl Pts',(-19.9532651082704,17.4782008180299,
-2.18902178704521));
#111070=CARTESIAN_POINT('Ctrl Pts',(-20.0231781449331,17.5295657222382,
-2.19476299579208));
#111071=CARTESIAN_POINT('Ctrl Pts',(-20.1737010323259,17.6550762826311,
-2.20752739975055));
#111072=CARTESIAN_POINT('Ctrl Pts',(-20.2521166851698,17.7314845843767,
-2.21446963224926));
#111073=CARTESIAN_POINT('Ctrl Pts',(-20.3336379992466,17.824259982578,-2.22200948829987));
#111074=CARTESIAN_POINT('Ctrl Pts',(-20.3428801360305,17.834993340225,-2.2228697172755));
#111075=CARTESIAN_POINT('Ctrl Pts',(-20.3574425044958,17.8522526736318,
-2.22423411278676));
#111076=CARTESIAN_POINT('Ctrl Pts',(-20.3628326070596,17.8587188888056,
-2.224741142035));
#111077=CARTESIAN_POINT('Ctrl Pts',(-20.3722848375392,17.8701967319361,
-2.22563392778639));
#111078=CARTESIAN_POINT('Ctrl Pts',(-20.3763628695648,17.8751950671355,
-2.22602032845939));
#111079=CARTESIAN_POINT('Ctrl Pts',(-20.3847637490828,17.8855884277285,
-2.22681890836706));
#111080=CARTESIAN_POINT('Ctrl Pts',(-20.3890831490421,17.8909861505662,
-2.22723094589812));
#111081=CARTESIAN_POINT('Ctrl Pts',(-20.4001304916741,17.9049308984128,
-2.22828856940508));
#111082=CARTESIAN_POINT('Ctrl Pts',(-20.4068191954625,17.9135088596134,
-2.2289325857393));
#111083=CARTESIAN_POINT('Ctrl Pts',(-20.4346932866237,17.9498299801156,
-2.23163248749914));
#111084=CARTESIAN_POINT('Ctrl Pts',(-20.4552576598895,17.9780443036075,
-2.2336639492588));
#111085=CARTESIAN_POINT('Ctrl Pts',(-20.5324401683793,18.089636002645,-2.24146597766943));
#111086=CARTESIAN_POINT('Ctrl Pts',(-20.5837764500916,18.1765077105203,
-2.24704183883486));
#111087=CARTESIAN_POINT('Ctrl Pts',(-20.6636064468633,18.3366885048602,
-2.25681069373311));
#111088=CARTESIAN_POINT('Ctrl Pts',(-20.6945765374082,18.4085405953949,
-2.26102810748162));
#111089=CARTESIAN_POINT('Ctrl Pts',(-20.7218617307922,18.4829231940916,
-2.26535938548301));
#111090=CARTESIAN_POINT('Ctrl Pts',(-20.7222215396299,18.4839063297364,
-2.26541662762247));
#111091=CARTESIAN_POINT('Ctrl Pts',(-20.7225806137756,18.4848897173872,
-2.26547387919804));
#111092=CARTESIAN_POINT('Ctrl Pts',(-20.7225806143688,18.484889719012,-2.04625075898636));
#111093=CARTESIAN_POINT('Ctrl Pts',(-20.7190678452871,18.4752693835319,
-2.0456673946269));
#111094=CARTESIAN_POINT('Ctrl Pts',(-20.7154851171429,18.4656741356815,
-2.04508128329489));
#111095=CARTESIAN_POINT('Ctrl Pts',(-20.7008063082509,18.4272155179506,
-2.04271348048677));
#111096=CARTESIAN_POINT('Ctrl Pts',(-20.6891489412846,18.3985730439432,
-2.04090771294304));
#111097=CARTESIAN_POINT('Ctrl Pts',(-20.6740381885879,18.3636561288022,
-2.03864182751629));
#111098=CARTESIAN_POINT('Ctrl Pts',(-20.6711741840977,18.3571288232929,
-2.03821543231835));
#111099=CARTESIAN_POINT('Ctrl Pts',(-20.6666170559015,18.3468836863867,
-2.03754154370128));
#111100=CARTESIAN_POINT('Ctrl Pts',(-20.6649460109763,18.3431560104146,
-2.03729538221779));
#111101=CARTESIAN_POINT('Ctrl Pts',(-20.6617920753989,18.3361745888825,
-2.03683249527082));
#111102=CARTESIAN_POINT('Ctrl Pts',(-20.6603117270573,18.3329197557002,
-2.03661592599276));
#111103=CARTESIAN_POINT('Ctrl Pts',(-20.6568999795337,18.3254685161816,
-2.03611839220421));
#111104=CARTESIAN_POINT('Ctrl Pts',(-20.6549630915615,18.3212746828098,
-2.03583709280961));
#111105=CARTESIAN_POINT('Ctrl Pts',(-20.6489187114161,18.3082988735045,
-2.03496288620491));
#111106=CARTESIAN_POINT('Ctrl Pts',(-20.6447646742806,18.2995388947276,
-2.03436721312599));
#111107=CARTESIAN_POINT('Ctrl Pts',(-20.5974955275657,18.2016017030713,
-2.02764827948139));
#111108=CARTESIAN_POINT('Ctrl Pts',(-20.5482373920097,18.115537297651,-2.021195611675));
#111109=CARTESIAN_POINT('Ctrl Pts',(-20.399449731234,17.8933013163034,-2.0035776289607));
#111110=CARTESIAN_POINT('Ctrl Pts',(-20.2893723145285,17.765010224037,-1.99238949452662));
#111111=CARTESIAN_POINT('Ctrl Pts',(-20.1423767404648,17.6301373120347,
-1.9798625993034));
#111112=CARTESIAN_POINT('Ctrl Pts',(-20.1190530915225,17.6096630672868,
-1.97793392486713));
#111113=CARTESIAN_POINT('Ctrl Pts',(-20.0836920553102,17.5799728486222,
-1.97509534439942));
#111114=CARTESIAN_POINT('Ctrl Pts',(-20.0719930233165,17.5703620445284,
-1.97416961807476));
#111115=CARTESIAN_POINT('Ctrl Pts',(-20.0530918684216,17.5551713226938,
-1.9726950683028));
#111116=CARTESIAN_POINT('Ctrl Pts',(-20.04595524529,17.5495110881048,-1.9721430324799));
#111117=CARTESIAN_POINT('Ctrl Pts',(-20.0322741886686,17.5388034115547,
-1.97109364827273));
#111118=CARTESIAN_POINT('Ctrl Pts',(-20.0257363115092,17.5337479009031,
-1.97059598362392));
#111119=CARTESIAN_POINT('Ctrl Pts',(-20.0142087486863,17.52494142388,-1.96972510511618));
#111120=CARTESIAN_POINT('Ctrl Pts',(-20.0092317974269,17.5211740248042,
-1.96935124475302));
#111121=CARTESIAN_POINT('Ctrl Pts',(-19.9993762615517,17.513782025418,-1.96861508121863));
#111122=CARTESIAN_POINT('Ctrl Pts',(-19.9944985893209,17.5101563140465,
-1.96825273668805));
#111123=CARTESIAN_POINT('Ctrl Pts',(-19.9827961448665,17.5015355474121,
-1.96738812041314));
#111124=CARTESIAN_POINT('Ctrl Pts',(-19.9759568870928,17.496560260653,-1.96688661920639));
#111125=CARTESIAN_POINT('Ctrl Pts',(-19.9511416912045,17.4787346163345,
-1.96508050613971));
#111126=CARTESIAN_POINT('Ctrl Pts',(-19.9329942545738,17.4661246211756,
-1.96378511870904));
#111127=CARTESIAN_POINT('Ctrl Pts',(-19.7605673997803,17.3502719999949,
-1.95170323482904));
#111128=CARTESIAN_POINT('Ctrl Pts',(-19.5935406163916,17.2674606365657,
-1.94177388522409));
#111129=CARTESIAN_POINT('Ctrl Pts',(-19.3420213280998,17.1816115205769,
-1.92728568526151));
#111130=CARTESIAN_POINT('Ctrl Pts',(-19.2647982366149,17.1600590543207,
-1.92287977218364));
#111131=CARTESIAN_POINT('Ctrl Pts',(-19.1513562354283,17.1352349761077,
-1.91623718674218));
#111132=CARTESIAN_POINT('Ctrl Pts',(-19.1159773718957,17.1284343706335,
-1.91414184751537));
#111133=CARTESIAN_POINT('Ctrl Pts',(-19.0730795303477,17.1213182513299,
-1.91155406408531));
#111134=CARTESIAN_POINT('Ctrl Pts',(-19.0657080621816,17.1201354667644,
-1.91110771450358));
#111135=CARTESIAN_POINT('Ctrl Pts',(-19.0542204789755,17.1183545106463,
-1.91040931555447));
#111136=CARTESIAN_POINT('Ctrl Pts',(-19.0501085126652,17.117729423413,-1.91015876392219));
#111137=CARTESIAN_POINT('Ctrl Pts',(-19.0424677606854,17.1165909290181,
-1.90969211006112));
#111138=CARTESIAN_POINT('Ctrl Pts',(-19.0389395103124,17.1160743186361,
-1.90947619137495));
#111139=CARTESIAN_POINT('Ctrl Pts',(-19.0309451845286,17.114924403995,-1.90898598685904));
#111140=CARTESIAN_POINT('Ctrl Pts',(-19.0264784026677,17.114296461136,-1.90871140344036));
#111141=CARTESIAN_POINT('Ctrl Pts',(-19.0149395420422,17.1127119112403,
-1.90800037643951));
#111142=CARTESIAN_POINT('Ctrl Pts',(-19.007864638088,17.1117767897605,-1.90756276579224));
#111143=CARTESIAN_POINT('Ctrl Pts',(-18.9643760245005,17.1062522925866,
-1.90486323660953));
#111144=CARTESIAN_POINT('Ctrl Pts',(-18.9278551237891,17.1025750331161,
-1.9025550410228));
#111145=CARTESIAN_POINT('Ctrl Pts',(-18.7213642553807,17.0871935138433,
-1.88934038092808));
#111146=CARTESIAN_POINT('Ctrl Pts',(-18.5505639565763,17.0950916986026,
-1.87784520490375));
#111147=CARTESIAN_POINT('Ctrl Pts',(-18.2884010190126,17.1392262784515,
-1.86056765255793));
#111148=CARTESIAN_POINT('Ctrl Pts',(-18.1954197599543,17.1614292173261,
-1.85450128655694));
#111149=CARTESIAN_POINT('Ctrl Pts',(-18.0838103250555,17.1962046114691,
-1.84732045803713));
#111150=CARTESIAN_POINT('Ctrl Pts',(-18.0634738039575,17.2028810432982,
-1.84601587830353));
#111151=CARTESIAN_POINT('Ctrl Pts',(-18.034722933616,17.2128053660157,-1.84417642340332));
#111152=CARTESIAN_POINT('Ctrl Pts',(-18.026223205722,17.2158002044253,-1.84363323020972));
#111153=CARTESIAN_POINT('Ctrl Pts',(-18.0116009287435,17.2210574932488,
-1.84269974419708));
#111154=CARTESIAN_POINT('Ctrl Pts',(-18.0054692935604,17.2232941340372,
-1.84230859983062));
#111155=CARTESIAN_POINT('Ctrl Pts',(-17.9937543168371,17.2276289045175,
-1.84156182444511));
#111156=CARTESIAN_POINT('Ctrl Pts',(-17.9881693159729,17.2297223400741,
-1.84120604126877));
#111157=CARTESIAN_POINT('Ctrl Pts',(-17.9736813109815,17.2352228463991,
-1.8402836761945));
#111158=CARTESIAN_POINT('Ctrl Pts',(-17.9647922757975,17.2386665213237,
-1.8397183250998));
#111159=CARTESIAN_POINT('Ctrl Pts',(-17.9346218912784,17.2505897309601,
-1.8378011256372));
#111160=CARTESIAN_POINT('Ctrl Pts',(-17.9134545780258,17.259354782647,-1.836458887937));
#111161=CARTESIAN_POINT('Ctrl Pts',(-17.7304096863751,17.3386554305616,
-1.82486619276819));
#111162=CARTESIAN_POINT('Ctrl Pts',(-17.5778061498537,17.428841159686,-1.81537759335669));
#111163=CARTESIAN_POINT('Ctrl Pts',(-17.3699643020394,17.5897248764056,
-1.80107399983594));
#111164=CARTESIAN_POINT('Ctrl Pts',(-17.3050623933915,17.6466274812604,
-1.79635040402545));
#111165=CARTESIAN_POINT('Ctrl Pts',(-17.2170891575077,17.7338113009417,
-1.78927749720031));
#111166=CARTESIAN_POINT('Ctrl Pts',(-17.1910744509895,17.7610050643575,
-1.78709140170358));
#111167=CARTESIAN_POINT('Ctrl Pts',(-17.1607210687907,17.7944762382524,
-1.78440297493004));
#111168=CARTESIAN_POINT('Ctrl Pts',(-17.155672242358,17.8001039554484,-1.78395102770745));
#111169=CARTESIAN_POINT('Ctrl Pts',(-17.1478792023388,17.8088847099593,
-1.78324576055274));
#111170=CARTESIAN_POINT('Ctrl Pts',(-17.1451139405222,17.8120190992573,
-1.78299398637949));
#111171=CARTESIAN_POINT('Ctrl Pts',(-17.1400081157992,17.8178411522909,
-1.7825262378712));
#111172=CARTESIAN_POINT('Ctrl Pts',(-17.1376650504122,17.8205265446659,
-1.78231045455948));
#111173=CARTESIAN_POINT('Ctrl Pts',(-17.132389860561,17.826603358792,-1.78182207696554));
#111174=CARTESIAN_POINT('Ctrl Pts',(-17.1294617383689,17.8299981661678,
-1.78154919457091));
#111175=CARTESIAN_POINT('Ctrl Pts',(-17.120869946294,17.8400235334818,-1.7807432512955));
#111176=CARTESIAN_POINT('Ctrl Pts',(-17.1152365164015,17.8466797223251,
-1.78020805361927));
#111177=CARTESIAN_POINT('Ctrl Pts',(-17.075428506715,17.8943085894367,-1.77637885816132));
#111178=CARTESIAN_POINT('Ctrl Pts',(-17.0427753817604,17.9365220978506,
-1.77298776242021));
#111179=CARTESIAN_POINT('Ctrl Pts',(-17.0014688792481,17.9943086844479,
-1.76839701273352));
#111180=CARTESIAN_POINT('Ctrl Pts',(-16.9913642515662,18.0088259421183,
-1.76724780278229));
#111181=CARTESIAN_POINT('Ctrl Pts',(-16.9542796703162,18.0635552758287,
-1.76293490378192));
#111182=CARTESIAN_POINT('Ctrl Pts',(-16.9285005056758,18.1045619374357,
-1.75974265646073));
#111183=CARTESIAN_POINT('Ctrl Pts',(-16.8491452090389,18.2409608759958,
-1.74931858448016));
#111184=CARTESIAN_POINT('Ctrl Pts',(-16.8015456967016,18.3396347972161,
-1.74208581379438));
#111185=CARTESIAN_POINT('Ctrl Pts',(-16.741756468379,18.4928838200185,-1.73151221537489));
#111186=CARTESIAN_POINT('Ctrl Pts',(-16.7237398247873,18.5449819925373,
-1.7280230083582));
#111187=CARTESIAN_POINT('Ctrl Pts',(-16.697838083891,18.630560181972,-1.72246534820155));
#111188=CARTESIAN_POINT('Ctrl Pts',(-16.6886997835665,18.6636308631711,
-1.72035845383858));
#111189=CARTESIAN_POINT('Ctrl Pts',(-16.6777441101147,18.7073954565616,
-1.71762190105163));
#111190=CARTESIAN_POINT('Ctrl Pts',(-16.6751997173642,18.7179003915396,
-1.71696890022378));
#111191=CARTESIAN_POINT('Ctrl Pts',(-16.6711634515564,18.7351408236112,
-1.71590340947858));
#111192=CARTESIAN_POINT('Ctrl Pts',(-16.669623873787,18.7418648461031,-1.71548939009587));
#111193=CARTESIAN_POINT('Ctrl Pts',(-16.6667068922995,18.7548970567613,
-1.71468988721327));
#111194=CARTESIAN_POINT('Ctrl Pts',(-16.6653254310474,18.7612042494961,
-1.71430427736103));
#111195=CARTESIAN_POINT('Ctrl Pts',(-16.6622017480666,18.7757845583152,
-1.71341587634844));
#111196=CARTESIAN_POINT('Ctrl Pts',(-16.6604801797879,18.7840620235377,
-1.71291375121927));
#111197=CARTESIAN_POINT('Ctrl Pts',(-16.6559824231989,18.8063567809199,
-1.71156718170263));
#111198=CARTESIAN_POINT('Ctrl Pts',(-16.6532984614739,18.8203923877775,
-1.71072567854518));
#111199=CARTESIAN_POINT('Ctrl Pts',(-16.6299799312036,18.9494024324239,
-1.70304537508105));
#111200=CARTESIAN_POINT('Ctrl Pts',(-16.6187508089804,19.0658798497603,
-1.69652311331571));
#111201=CARTESIAN_POINT('Ctrl Pts',(-16.6150144979993,19.3453779252748,
-1.68122065926736));
#111202=CARTESIAN_POINT('Ctrl Pts',(-16.6315990743005,19.5077414717001,
-1.67262337881141));
#111203=CARTESIAN_POINT('Ctrl Pts',(-16.6736115328653,19.6983901181167,
-1.66141475394752));
#111204=CARTESIAN_POINT('Ctrl Pts',(-16.6813531724137,19.7300284204965,
-1.65951524838366));
#111205=CARTESIAN_POINT('Ctrl Pts',(-16.6917045230492,19.7684680761476,
-1.65714500416665));
#111206=CARTESIAN_POINT('Ctrl Pts',(-16.693623922798,19.7754527714791,-1.65671177622824));
#111207=CARTESIAN_POINT('Ctrl Pts',(-16.6966886322803,19.7863853383506,
-1.65602949294841));
#111208=CARTESIAN_POINT('Ctrl Pts',(-16.6978096797495,19.7903400345965,
-1.65578182540814));
#111209=CARTESIAN_POINT('Ctrl Pts',(-16.6999263418473,19.7977249019883,
-1.65531768475457));
#111210=CARTESIAN_POINT('Ctrl Pts',(-16.7009191219703,19.8011558269973,
-1.65510137735003));
#111211=CARTESIAN_POINT('Ctrl Pts',(-16.7032047709694,19.8089805301996,
-1.65460652994716));
#111212=CARTESIAN_POINT('Ctrl Pts',(-16.7045032144444,19.8133726199457,
-1.65432766855632));
#111213=CARTESIAN_POINT('Ctrl Pts',(-16.7085367007406,19.8268551290962,
-1.65346833805376));
#111214=CARTESIAN_POINT('Ctrl Pts',(-16.7113186002461,19.8359312474635,
-1.652885234344));
#111215=CARTESIAN_POINT('Ctrl Pts',(-16.7367835368353,19.9170606218719,
-1.64763344775525));
#111216=CARTESIAN_POINT('Ctrl Pts',(-16.7632447056273,19.9878630869451,
-1.64277153447652));
#111217=CARTESIAN_POINT('Ctrl Pts',(-16.8475448761804,20.1812114853825,
-1.62897837287824));
#111218=CARTESIAN_POINT('Ctrl Pts',(-16.9134494627898,20.2998630218719,
-1.61992773292954));
#111219=CARTESIAN_POINT('Ctrl Pts',(-17.0412259322724,20.4854769435079,
-1.60532414890131));
#111220=CARTESIAN_POINT('Ctrl Pts',(-17.0968888214295,20.5562308769006,
-1.59962552812818));
#111221=CARTESIAN_POINT('Ctrl Pts',(-17.1707195242886,20.6386809476795,
-1.59283182932643));
#111222=CARTESIAN_POINT('Ctrl Pts',(-17.1847748556969,20.6539207304438,
-1.59156881984961));
#111223=CARTESIAN_POINT('Ctrl Pts',(-17.2051793221326,20.6754027754882,
-1.58977737081244));
#111224=CARTESIAN_POINT('Ctrl Pts',(-17.2113471489855,20.681814894202,-1.58924119213932));
#111225=CARTESIAN_POINT('Ctrl Pts',(-17.2220950721111,20.6928484464511,
-1.58831596558539));
#111226=CARTESIAN_POINT('Ctrl Pts',(-17.2266563535593,20.6974879623549,
-1.58792610574032));
#111227=CARTESIAN_POINT('Ctrl Pts',(-17.2354573882277,20.7063577865244,
-1.58717917307284));
#111228=CARTESIAN_POINT('Ctrl Pts',(-17.2396938407051,20.7105912684611,
-1.58682196062898));
#111229=CARTESIAN_POINT('Ctrl Pts',(-17.250815938143,20.7216116345574,-1.58589018190079));
#111230=CARTESIAN_POINT('Ctrl Pts',(-17.2577302605293,20.7283694780248,
-1.58531689756478));
#111231=CARTESIAN_POINT('Ctrl Pts',(-17.2817714603034,20.7515467143845,
-1.58334382810852));
#111232=CARTESIAN_POINT('Ctrl Pts',(-17.2991282910977,20.7677257807722,
-1.5819544402883));
#111233=CARTESIAN_POINT('Ctrl Pts',(-17.4372178387847,20.8921729389442,
-1.57116043397875));
#111234=CARTESIAN_POINT('Ctrl Pts',(-17.5697566900678,20.9865367991548,
-1.56238143124986));
#111235=CARTESIAN_POINT('Ctrl Pts',(-17.8259908979364,21.1278249193074,
-1.54648533972015));
#111236=CARTESIAN_POINT('Ctrl Pts',(-17.9457581808062,21.1801021444401,
-1.53939274147877));
#111237=CARTESIAN_POINT('Ctrl Pts',(-18.0808430655757,21.2247567998446,
-1.53099669199578));
#111238=CARTESIAN_POINT('Ctrl Pts',(-18.0921655107044,21.2283940873398,
-1.53028995139147));
#111239=CARTESIAN_POINT('Ctrl Pts',(-18.1083098766694,21.2334307329601,
-1.52927717034302));
#111240=CARTESIAN_POINT('Ctrl Pts',(-18.1131072948517,21.234908705344,-1.52897558269147));
#111241=CARTESIAN_POINT('Ctrl Pts',(-18.1213857646729,21.2374269042973,
-1.52845399910139));
#111242=CARTESIAN_POINT('Ctrl Pts',(-18.1248643571753,21.2384752694612,
-1.52823447783377));
#111243=CARTESIAN_POINT('Ctrl Pts',(-18.1316159470946,21.2404910941323,
-1.52780769857028));
#111244=CARTESIAN_POINT('Ctrl Pts',(-18.1348885920772,21.2414595954786,
-1.52760050881988));
#111245=CARTESIAN_POINT('Ctrl Pts',(-18.1437278408755,21.2440522382063,
-1.52704006298681));
#111246=CARTESIAN_POINT('Ctrl Pts',(-18.1492987512022,21.2456614148179,
-1.5266859493317));
#111247=CARTESIAN_POINT('Ctrl Pts',(-18.170019326319,21.2515544994108,-1.52536571578831));
#111248=CARTESIAN_POINT('Ctrl Pts',(-18.1852095920935,21.2556921332941,
-1.52439164039854));
#111249=CARTESIAN_POINT('Ctrl Pts',(-18.32787796054,21.2928488899631,-1.51519416206896));
#111250=CARTESIAN_POINT('Ctrl Pts',(-18.4581190231792,21.3140723916972,
-1.50645220198235));
#111251=CARTESIAN_POINT('Ctrl Pts',(-18.7483780155742,21.3339345601522,
-1.48723402036962));
#111252=CARTESIAN_POINT('Ctrl Pts',(-18.9080304619821,21.3268424909805,
-1.47686494019605));
#111253=CARTESIAN_POINT('Ctrl Pts',(-19.0864174680456,21.2985688712288,
-1.46577189765157));
#111254=CARTESIAN_POINT('Ctrl Pts',(-19.1073848533288,21.29492074396,-1.46447486056233));
#111255=CARTESIAN_POINT('Ctrl Pts',(-19.137128302477,21.2892823234735,-1.46264408471769));
#111256=CARTESIAN_POINT('Ctrl Pts',(-19.1459516656374,21.2875513895393,
-1.46210213502894));
#111257=CARTESIAN_POINT('Ctrl Pts',(-19.1611569950002,21.2844677366788,
-1.46117009979723));
#111258=CARTESIAN_POINT('Ctrl Pts',(-19.1675441768289,21.2831416461337,
-1.46077916987309));
#111259=CARTESIAN_POINT('Ctrl Pts',(-19.17976391058,21.2805456422496,-1.46003233689425));
#111260=CARTESIAN_POINT('Ctrl Pts',(-19.185597411166,21.2792805439983,-1.45967628392075));
#111261=CARTESIAN_POINT('Ctrl Pts',(-19.2007567509899,21.2759257786496,
-1.45875220920336));
#111262=CARTESIAN_POINT('Ctrl Pts',(-19.2100739958683,21.2737975884552,
-1.45818542731458));
#111263=CARTESIAN_POINT('Ctrl Pts',(-19.2418174444575,21.2663204067912,
-1.45625818626532));
#111264=CARTESIAN_POINT('Ctrl Pts',(-19.264171028183,21.2606680886822,-1.45490747644726));
#111265=CARTESIAN_POINT('Ctrl Pts',(-19.4549968071667,21.2090851292604,
-1.44342161133107));
#111266=CARTESIAN_POINT('Ctrl Pts',(-19.6172786135118,21.1428401096183,
-1.43402871203011));
#111267=CARTESIAN_POINT('Ctrl Pts',(-19.846006883766,21.0145535142479,-1.41976145696229));
#111268=CARTESIAN_POINT('Ctrl Pts',(-19.9196792641771,20.9669973918359,
-1.41496702939098));
#111269=CARTESIAN_POINT('Ctrl Pts',(-20.0207558050714,20.8924846767388,
-1.40779861654817));
#111270=CARTESIAN_POINT('Ctrl Pts',(-20.0507099584124,20.8691331978145,
-1.40559291803075));
#111271=CARTESIAN_POINT('Ctrl Pts',(-20.0858687956549,20.8401707167837,
-1.4028827589211));
#111272=CARTESIAN_POINT('Ctrl Pts',(-20.0916937734104,20.8353195740972,
-1.40242963365393));
#111273=CARTESIAN_POINT('Ctrl Pts',(-20.1006932920051,20.8277423893667,
-1.40172291874549));
#111274=CARTESIAN_POINT('Ctrl Pts',(-20.1038860843742,20.8250379868916,
-1.40147088500506));
#111275=CARTESIAN_POINT('Ctrl Pts',(-20.1097830276902,20.8200129764703,
-1.40100291356065));
#111276=CARTESIAN_POINT('Ctrl Pts',(-20.1124893449939,20.817694999959,-1.40078716852823));
#111277=CARTESIAN_POINT('Ctrl Pts',(-20.1185827513068,20.812449233957,-1.40029920425895));
#111278=CARTESIAN_POINT('Ctrl Pts',(-20.1219663921994,20.809517543673,-1.40002669898897));
#111279=CARTESIAN_POINT('Ctrl Pts',(-20.1318927159867,20.8008617948016,
-1.39922279338479));
#111280=CARTESIAN_POINT('Ctrl Pts',(-20.1384093776285,20.7951082242273,
-1.39868927156008));
#111281=CARTESIAN_POINT('Ctrl Pts',(-20.1842710770323,20.7541114430327,
-1.39489478221264));
#111282=CARTESIAN_POINT('Ctrl Pts',(-20.2223171047442,20.7174495705688,
-1.39153861526006));
#111283=CARTESIAN_POINT('Ctrl Pts',(-20.2724917413791,20.6653429351066,
-1.38686514685341));
#111284=CARTESIAN_POINT('Ctrl Pts',(-20.2858390408807,20.651092278134,-1.38559624224201));
#111285=CARTESIAN_POINT('Ctrl Pts',(-20.3975968402582,20.5284125485089,
-1.37476366487907));
#111286=CARTESIAN_POINT('Ctrl Pts',(-20.4847193863943,20.4102152054933,
-1.36495843767335));
#111287=CARTESIAN_POINT('Ctrl Pts',(-20.5902290357467,20.2307612337731,
-1.35150939859198));
#111288=CARTESIAN_POINT('Ctrl Pts',(-20.6191743012523,20.1762037026442,
-1.347583287487));
#111289=CARTESIAN_POINT('Ctrl Pts',(-20.6616864783605,20.0868420836187,
-1.34141728728218));
#111290=CARTESIAN_POINT('Ctrl Pts',(-20.6767885689105,20.0528119545064,
-1.33912762571612));
#111291=CARTESIAN_POINT('Ctrl Pts',(-20.6952311505789,20.0081105667389,
-1.33619305310821));
#111292=CARTESIAN_POINT('Ctrl Pts',(-20.6993949396811,19.9977881672321,
-1.33552036370463));
#111293=CARTESIAN_POINT('Ctrl Pts',(-20.7060329042927,19.980950506244,-1.33443100152554));
#111294=CARTESIAN_POINT('Ctrl Pts',(-20.7085566179745,19.9744551210768,
-1.33401266450816));
#111295=CARTESIAN_POINT('Ctrl Pts',(-20.7133473849458,19.9619422592231,
-1.3332103758235));
#111296=CARTESIAN_POINT('Ctrl Pts',(-20.7156191794287,19.9559266917677,
-1.33282626855246));
#111297=CARTESIAN_POINT('Ctrl Pts',(-20.7207568627085,19.9421326041437,
-1.33194908268649));
#111298=CARTESIAN_POINT('Ctrl Pts',(-20.7236045542558,19.9343473833711,
-1.33145661645791));
#111299=CARTESIAN_POINT('Ctrl Pts',(-20.7310458706766,19.9136273509501,
-1.33015272451114));
#111300=CARTESIAN_POINT('Ctrl Pts',(-20.7355595981026,19.9006641156193,
-1.32934395282688));
#111301=CARTESIAN_POINT('Ctrl Pts',(-20.7688588159741,19.8019488125391,
-1.32323618964279));
#111302=CARTESIAN_POINT('Ctrl Pts',(-20.7922498000777,19.7144695028033,
-1.31812049820499));
#111303=CARTESIAN_POINT('Ctrl Pts',(-20.8373639130496,19.4886586124642,
-1.3053742556948));
#111304=CARTESIAN_POINT('Ctrl Pts',(-20.8511051845503,19.3491947094905,
-1.29793919539568));
#111305=CARTESIAN_POINT('Ctrl Pts',(-20.8509840406832,19.1891096026292,
-1.28909428040406));
#111306=CARTESIAN_POINT('Ctrl Pts',(-20.8506770365379,19.1688228885415,
-1.28796720666155));
#111307=CARTESIAN_POINT('Ctrl Pts',(-20.8483264336703,19.0891816749561,
-1.28350793907996));
#111308=CARTESIAN_POINT('Ctrl Pts',(-20.8440773401239,19.029924794281,-1.28011469178611));
#111309=CARTESIAN_POINT('Ctrl Pts',(-20.8363297207849,18.9620447043256,
-1.27606213717897));
#111310=CARTESIAN_POINT('Ctrl Pts',(-20.8352591883989,18.9531651479409,
-1.27552872938984));
#111311=CARTESIAN_POINT('Ctrl Pts',(-20.8335616374147,18.9397981216427,
-1.27472044424236));
#111312=CARTESIAN_POINT('Ctrl Pts',(-20.8329764096806,18.9353053158733,
-1.2744478656179));
#111313=CARTESIAN_POINT('Ctrl Pts',(-20.8319046586927,18.9272787151137,
-1.27395921812067));
#111314=CARTESIAN_POINT('Ctrl Pts',(-20.831423622613,18.9237442402599,-1.27374346151846));
#111315=CARTESIAN_POINT('Ctrl Pts',(-20.8303644473174,18.9161063311495,
-1.2732759425222));
#111316=CARTESIAN_POINT('Ctrl Pts',(-20.8297832003396,18.9120034307911,
-1.2730240118858));
#111317=CARTESIAN_POINT('Ctrl Pts',(-20.8281309513191,18.9005821117377,
-1.27232055547921));
#111318=CARTESIAN_POINT('Ctrl Pts',(-20.827033648108,18.8932676428192,-1.2718675827939));
#111319=CARTESIAN_POINT('Ctrl Pts',(-20.8205389576268,18.8514691043742,
-1.26926555580998));
#111320=CARTESIAN_POINT('Ctrl Pts',(-20.8143280450887,18.817119074259,-1.26707459920712));
#111321=CARTESIAN_POINT('Ctrl Pts',(-20.7918958078795,18.7084703106017,
-1.26000962832172));
#111322=CARTESIAN_POINT('Ctrl Pts',(-20.7725200131397,18.634887319593,-1.25502398948114));
#111323=CARTESIAN_POINT('Ctrl Pts',(-20.7408447834904,18.5364539837809,
-1.2482018376817));
#111324=CARTESIAN_POINT('Ctrl Pts',(-20.7319594999981,18.5105754523218,
-1.24639321905346));
#111325=CARTESIAN_POINT('Ctrl Pts',(-20.7225806756345,18.4848898867987,
-1.24458630806144));
#111326=CARTESIAN_POINT('Origin',(-18.734,19.211,0.));
#111327=CARTESIAN_POINT('',(-20.7225806137986,18.4848897174502,-0.444429630404752));
#111328=CARTESIAN_POINT('',(-20.7225806137986,18.4848897174502,-0.666446459697765));
#111329=CARTESIAN_POINT('',(-20.7225806137986,18.4848897174502,0.));
#111330=CARTESIAN_POINT('',(-17.1140743056112,20.5739122292573,0.));
#111331=CARTESIAN_POINT('Ctrl Pts',(-20.7225806137986,18.4848897174502,
-0.444429630404752));
#111332=CARTESIAN_POINT('Ctrl Pts',(-20.6978891218494,18.4172677275186,
-0.44011526652472));
#111333=CARTESIAN_POINT('Ctrl Pts',(-20.6697399412968,18.3508947277507,
-0.435800902644688));
#111334=CARTESIAN_POINT('Ctrl Pts',(-20.6382938060541,18.2861464439036,
-0.431486538764656));
#111335=CARTESIAN_POINT('Ctrl Pts',(-20.6068209811841,18.2213432055274,
-0.427168513106713));
#111336=CARTESIAN_POINT('Ctrl Pts',(-20.5720458283503,18.1581678859396,
-0.422850487448771));
#111337=CARTESIAN_POINT('Ctrl Pts',(-20.5341758800126,18.0969731596496,
-0.418532461790828));
#111338=CARTESIAN_POINT('Ctrl Pts',(-20.496290462457,18.0357534363742,-0.414212672294214));
#111339=CARTESIAN_POINT('Ctrl Pts',(-20.4553080152584,17.9765163262865,
-0.4098928827976));
#111340=CARTESIAN_POINT('Ctrl Pts',(-20.4114788156669,17.9195845660715,
-0.405573093300986));
#111341=CARTESIAN_POINT('Ctrl Pts',(-20.3675728424278,17.8625530810398,
-0.401245737022412));
#111342=CARTESIAN_POINT('Ctrl Pts',(-20.3208104807034,17.8078353893813,
-0.396918380743837));
#111343=CARTESIAN_POINT('Ctrl Pts',(-20.2714811519989,17.7557197152273,
-0.392591024465263));
#111344=CARTESIAN_POINT('Ctrl Pts',(-20.2294416137679,17.7113055921575,
-0.388903156324941));
#111345=CARTESIAN_POINT('Ctrl Pts',(-20.1855385022242,17.6687807601312,
-0.385215288184619));
#111346=CARTESIAN_POINT('Ctrl Pts',(-20.139969531998,17.6283001942588,-0.381527420044297));
#111347=CARTESIAN_POINT('Ctrl Pts',(-20.0856806361702,17.5800734028086,
-0.377133853801673));
#111348=CARTESIAN_POINT('Ctrl Pts',(-20.028804456646,17.534551575879,-0.372740287559049));
#111349=CARTESIAN_POINT('Ctrl Pts',(-19.9696413059749,17.4920236874905,
-0.368346721316425));
#111350=CARTESIAN_POINT('Ctrl Pts',(-19.9105644543723,17.4495578329375,
-0.36395956380406));
#111351=CARTESIAN_POINT('Ctrl Pts',(-19.8492076419246,17.4100775251571,
-0.359572406291694));
#111352=CARTESIAN_POINT('Ctrl Pts',(-19.7859055363078,17.3738326851686,
-0.355185248779329));
#111353=CARTESIAN_POINT('Ctrl Pts',(-19.7226758978493,17.3376293376475,
-0.350803113609185));
#111354=CARTESIAN_POINT('Ctrl Pts',(-19.6575058056517,17.3046543374869,
-0.346420978439041));
#111355=CARTESIAN_POINT('Ctrl Pts',(-19.5907589079217,17.2751143696755,
-0.342038843268897));
#111356=CARTESIAN_POINT('Ctrl Pts',(-19.5240531514201,17.2455926096102,
-0.33765940914449));
#111357=CARTESIAN_POINT('Ctrl Pts',(-19.4557729567064,17.2195018746871,
-0.333279975020084));
#111358=CARTESIAN_POINT('Ctrl Pts',(-19.3863053176006,17.1970022908082,
-0.328900540895677));
#111359=CARTESIAN_POINT('Ctrl Pts',(-19.3168577535507,17.1745092089554,
-0.324522372358906));
#111360=CARTESIAN_POINT('Ctrl Pts',(-19.2462238836977,17.1556053656812,
-0.320144203822134));
#111361=CARTESIAN_POINT('Ctrl Pts',(-19.1748077989579,17.1404016602977,
-0.315766035285363));
#111362=CARTESIAN_POINT('Ctrl Pts',(-19.1033889720517,17.1251973711369,
-0.311387698639869));
#111363=CARTESIAN_POINT('Ctrl Pts',(-19.0311883413904,17.1136936001516,
-0.307009361994375));
#111364=CARTESIAN_POINT('Ctrl Pts',(-18.9586205452228,17.1059502118326,
-0.302631025348881));
#111365=CARTESIAN_POINT('Ctrl Pts',(-18.8859767969382,17.0981987189992,
-0.298248106175667));
#111366=CARTESIAN_POINT('Ctrl Pts',(-18.8129655950942,17.0942155178377,
-0.293865187002452));
#111367=CARTESIAN_POINT('Ctrl Pts',(-18.740006248305,17.0940085203333,-0.289482267829238));
#111368=CARTESIAN_POINT('Ctrl Pts',(-18.6670065469439,17.0938014083365,
-0.285096924417943));
#111369=CARTESIAN_POINT('Ctrl Pts',(-18.5940592383891,17.0973746352134,
-0.280711581006648));
#111370=CARTESIAN_POINT('Ctrl Pts',(-18.5215804684087,17.1046840354309,
-0.276326237595353));
#111371=CARTESIAN_POINT('Ctrl Pts',(-18.4489736078896,17.1120063534313,
-0.271933144038736));
#111372=CARTESIAN_POINT('Ctrl Pts',(-18.3768374152679,17.1230779575914,
-0.267540050482118));
#111373=CARTESIAN_POINT('Ctrl Pts',(-18.3055792094826,17.1378032832718,
-0.263146956925501));
#111374=CARTESIAN_POINT('Ctrl Pts',(-18.2580242315412,17.1476303976399,
-0.260215175737955));
#111375=CARTESIAN_POINT('Ctrl Pts',(-18.2108600441032,17.159083715391,-0.25728339455041));
#111376=CARTESIAN_POINT('Ctrl Pts',(-18.1642034381997,17.1721226426878,
-0.254351613362864));
#111377=CARTESIAN_POINT('Ctrl Pts',(-18.0951058972849,17.1914330446111,
-0.250009701502006));
#111378=CARTESIAN_POINT('Ctrl Pts',(-18.0268399854881,17.2143024101294,
-0.245667789641149));
#111379=CARTESIAN_POINT('Ctrl Pts',(-17.9598043906283,17.2406421242755,
-0.241325877780291));
#111380=CARTESIAN_POINT('Ctrl Pts',(-17.8928697395248,17.266942175468,-0.236990504071195));
#111381=CARTESIAN_POINT('Ctrl Pts',(-17.8271621848895,17.29670202984,-0.232655130362099));
#111382=CARTESIAN_POINT('Ctrl Pts',(-17.7630669345952,17.3297828454685,
-0.228319756653002));
#111383=CARTESIAN_POINT('Ctrl Pts',(-17.6990453506666,17.3628256404409,
-0.223989365703525));
#111384=CARTESIAN_POINT('Ctrl Pts',(-17.6366328289126,17.3991815955316,
-0.219658974754049));
#111385=CARTESIAN_POINT('Ctrl Pts',(-17.5761945067698,17.4386638468265,
-0.215328583804572));
#111386=CARTESIAN_POINT('Ctrl Pts',(-17.5157933283169,17.4781218334421,
-0.211000854191362));
#111387=CARTESIAN_POINT('Ctrl Pts',(-17.4573643561352,17.5207020380533,
-0.206673124578153));
#111388=CARTESIAN_POINT('Ctrl Pts',(-17.4012466091921,17.5661725320599,
-0.202345394964943));
#111389=CARTESIAN_POINT('Ctrl Pts',(-17.3451439091011,17.6116308340625,
-0.19801882574592));
#111390=CARTESIAN_POINT('Ctrl Pts',(-17.2913515880726,17.6599775776503,
-0.193692256526897));
#111391=CARTESIAN_POINT('Ctrl Pts',(-17.2401767514858,17.7109396338152,
-0.189365687307874));
#111392=CARTESIAN_POINT('Ctrl Pts',(-17.1889979072006,17.7619056810149,
-0.185038779258564));
#111393=CARTESIAN_POINT('Ctrl Pts',(-17.1404373022758,17.8154870975619,
-0.180711871209254));
#111394=CARTESIAN_POINT('Ctrl Pts',(-17.0947649174399,17.8713741775764,
-0.176384963159944));
#111395=CARTESIAN_POINT('Ctrl Pts',(-17.0490377231869,17.9273283252136,
-0.172052862578908));
#111396=CARTESIAN_POINT('Ctrl Pts',(-17.0062059805783,17.9855932764931,
-0.167720761997871));
#111397=CARTESIAN_POINT('Ctrl Pts',(-16.9664985330235,18.0458272384595,
-0.163388661416834));
#111398=CARTESIAN_POINT('Ctrl Pts',(-16.9267665792056,18.1060983750471,
-0.159053887191346));
#111399=CARTESIAN_POINT('Ctrl Pts',(-16.8901630045679,18.1683405133195,
-0.154719112965857));
#111400=CARTESIAN_POINT('Ctrl Pts',(-16.8568710208891,18.2321865367793,
-0.150384338740368));
#111401=CARTESIAN_POINT('Ctrl Pts',(-16.8235119906461,18.2961611394355,
-0.146040834734123));
#111402=CARTESIAN_POINT('Ctrl Pts',(-16.7934780711976,18.3617456271075,
-0.141697330727878));
#111403=CARTESIAN_POINT('Ctrl Pts',(-16.7669043702654,18.4285526960369,
-0.137353826721632));
#111404=CARTESIAN_POINT('Ctrl Pts',(-16.7461478827044,18.4807351187547,
-0.133961153374898));
#111405=CARTESIAN_POINT('Ctrl Pts',(-16.7275015133356,18.5336630097784,
-0.130568480028163));
#111406=CARTESIAN_POINT('Ctrl Pts',(-16.7110080390405,18.5871470318309,
-0.127175806681429));
#111407=CARTESIAN_POINT('Ctrl Pts',(-16.6890808417458,18.6582511959801,
-0.122665427818863));
#111408=CARTESIAN_POINT('Ctrl Pts',(-16.6708715522275,18.7306260888239,
-0.118155048956298));
#111409=CARTESIAN_POINT('Ctrl Pts',(-16.6565194459451,18.8038593025457,
-0.113644670093733));
#111410=CARTESIAN_POINT('Ctrl Pts',(-16.6414519720022,18.8807427590775,
-0.108909475506494));
#111411=CARTESIAN_POINT('Ctrl Pts',(-16.6306364414031,18.9585718864235,
-0.104174280919255));
#111412=CARTESIAN_POINT('Ctrl Pts',(-16.624175177866,19.0368500074442,-0.0994390863320157));
#111413=CARTESIAN_POINT('Ctrl Pts',(-16.6180411415214,19.1111637754199,
-0.094943703110145));
#111414=CARTESIAN_POINT('Ctrl Pts',(-16.6158311470803,19.18588164953,-0.0904483198882744));
#111415=CARTESIAN_POINT('Ctrl Pts',(-16.6175803959886,19.2605687376906,
-0.0859529366664038));
#111416=CARTESIAN_POINT('Ctrl Pts',(-16.6193280001048,19.3351855987192,
-0.0814617803849424));
#111417=CARTESIAN_POINT('Ctrl Pts',(-16.6250274372589,19.4097712832384,
-0.076970624103481));
#111418=CARTESIAN_POINT('Ctrl Pts',(-16.6346618981062,19.4838892338239,
-0.0724794678220196));
#111419=CARTESIAN_POINT('Ctrl Pts',(-16.6442898170097,19.5579568572063,
-0.0679913611032213));
#111420=CARTESIAN_POINT('Ctrl Pts',(-16.6578473889511,19.6315569329051,
-0.0635032543844231));
#111421=CARTESIAN_POINT('Ctrl Pts',(-16.6752659458499,19.7042576347942,
-0.0590151476656248));
#111422=CARTESIAN_POINT('Ctrl Pts',(-16.6926772219334,19.7769279483805,
-0.054528916938974));
#111423=CARTESIAN_POINT('Ctrl Pts',(-16.7139461674509,19.8486991989659,
-0.0500426862123233));
#111424=CARTESIAN_POINT('Ctrl Pts',(-16.7389532085404,19.9191506194918,
-0.0455564554856726));
#111425=CARTESIAN_POINT('Ctrl Pts',(-16.7639633583527,19.9896107981086,
-0.0410696670581851));
#111426=CARTESIAN_POINT('Ctrl Pts',(-16.7927123885946,20.0587503922126,
-0.0365828786306977));
#111427=CARTESIAN_POINT('Ctrl Pts',(-16.8250314087851,20.1261655138581,
-0.0320960902032102));
#111428=CARTESIAN_POINT('Ctrl Pts',(-16.8573519842581,20.1935838797095,
-0.0276090858587984));
#111429=CARTESIAN_POINT('Ctrl Pts',(-16.8932426902261,20.2592772053156,
-0.0231220815143867));
#111430=CARTESIAN_POINT('Ctrl Pts',(-16.9324879501579,20.3228648003574,
-0.0186350771699749));
#111431=CARTESIAN_POINT('Ctrl Pts',(-16.9717602972259,20.3864962836508,
-0.0141449758885697));
#111432=CARTESIAN_POINT('Ctrl Pts',(-17.0143915779344,20.4480187554703,
-0.00965487460716451));
#111433=CARTESIAN_POINT('Ctrl Pts',(-17.0601224600125,20.5070798513692,
-0.00516477332575931));
#111434=CARTESIAN_POINT('Ctrl Pts',(-17.0776565589201,20.5297250103958,
-0.0034431822171712));
#111435=CARTESIAN_POINT('Ctrl Pts',(-17.0956458992255,20.5520086551532,
-0.00172159110858308));
#111436=CARTESIAN_POINT('Ctrl Pts',(-17.1140743056112,20.5739122292573,
5.04250086090388E-15));
#111437=CARTESIAN_POINT('',(-20.3539402423909,20.5738949376539,-2.19221144982933E-7));
#111438=CARTESIAN_POINT('Origin',(-18.734,19.211,0.));
#111439=CARTESIAN_POINT('Ctrl Pts',(-20.3539402423909,20.5738949376539,
-2.19221144982933E-7));
#111440=CARTESIAN_POINT('Ctrl Pts',(-20.307293457224,20.6293394201171,-0.00438523054252598));
#111441=CARTESIAN_POINT('Ctrl Pts',(-20.2577052453279,20.6824952398001,
-0.00877024186390698));
#111442=CARTESIAN_POINT('Ctrl Pts',(-20.2054289850318,20.7330334234202,
-0.013155253185288));
#111443=CARTESIAN_POINT('Ctrl Pts',(-20.1532303457042,20.7834965668072,
-0.0175337535431148));
#111444=CARTESIAN_POINT('Ctrl Pts',(-20.0983519254295,20.8313494565076,
-0.0219122539009416));
#111445=CARTESIAN_POINT('Ctrl Pts',(-20.0410868627427,20.8762966502235,
-0.0262907542587684));
#111446=CARTESIAN_POINT('Ctrl Pts',(-19.9838891952347,20.9211909456447,
-0.0306641015651428));
#111447=CARTESIAN_POINT('Ctrl Pts',(-19.9243108432099,20.9631860414448,
-0.0350374488715171));
#111448=CARTESIAN_POINT('Ctrl Pts',(-19.8626799780619,21.0020249878553,
-0.0394107961778915));
#111449=CARTESIAN_POINT('Ctrl Pts',(-19.8010881104923,21.0408393585139,
-0.0437813762027535));
#111450=CARTESIAN_POINT('Ctrl Pts',(-19.7374467144136,21.0765012852422,
-0.0481519562276155));
#111451=CARTESIAN_POINT('Ctrl Pts',(-19.6721138966917,21.1087964371433,
-0.0525225362524776));
#111452=CARTESIAN_POINT('Ctrl Pts',(-19.606800782292,21.1410818493484,-0.0568917981810183));
#111453=CARTESIAN_POINT('Ctrl Pts',(-19.5397976918716,21.170002288633,-0.061261060109559));
#111454=CARTESIAN_POINT('Ctrl Pts',(-19.4714868524903,21.1953896145677,
-0.0656303220380997));
#111455=CARTESIAN_POINT('Ctrl Pts',(-19.4031739921601,21.2207776915762,
-0.069999713229504));
#111456=CARTESIAN_POINT('Ctrl Pts',(-19.3335537597041,21.2426322814668,
-0.0743691044209083));
#111457=CARTESIAN_POINT('Ctrl Pts',(-19.2630262593489,21.2608341925432,
-0.0787384956123125));
#111458=CARTESIAN_POINT('Ctrl Pts',(-19.1924269638888,21.2790546326772,
-0.0831123347268293));
#111459=CARTESIAN_POINT('Ctrl Pts',(-19.1209190256059,21.2936148503493,
-0.087486173841346));
#111460=CARTESIAN_POINT('Ctrl Pts',(-19.0489146836732,21.3044463790618,
-0.0918600129558628));
#111461=CARTESIAN_POINT('Ctrl Pts',(-18.9768705191302,21.3152838982429,
-0.0962362710591022));
#111462=CARTESIAN_POINT('Ctrl Pts',(-18.9043298854537,21.3223885760892,
-0.100612529162342));
#111463=CARTESIAN_POINT('Ctrl Pts',(-18.8317094286016,21.3257439248198,
-0.104988787265581));
#111464=CARTESIAN_POINT('Ctrl Pts',(-18.7589648320258,21.3291050092905,
-0.109372526283915));
#111465=CARTESIAN_POINT('Ctrl Pts',(-18.6861406230803,21.3287039714963,
-0.113756265302249));
#111466=CARTESIAN_POINT('Ctrl Pts',(-18.6136520423462,21.324576440323,-0.118140004320582));
#111467=CARTESIAN_POINT('Ctrl Pts',(-18.5716442693833,21.3221844995419,
-0.120680419811489));
#111468=CARTESIAN_POINT('Ctrl Pts',(-18.5297491060652,21.3185420587999,
-0.123220835302396));
#111469=CARTESIAN_POINT('Ctrl Pts',(-18.4880458562809,21.3136639196951,
-0.125761250793303));
#111470=CARTESIAN_POINT('Ctrl Pts',(-18.415885212538,21.3052230988983,-0.13015702374017));
#111471=CARTESIAN_POINT('Ctrl Pts',(-18.3440242467257,21.2930474771355,
-0.134552796687037));
#111472=CARTESIAN_POINT('Ctrl Pts',(-18.2728788054799,21.2771694615796,
-0.138948569633904));
#111473=CARTESIAN_POINT('Ctrl Pts',(-18.2018361910671,21.2613143945926,
-0.143337989349932));
#111474=CARTESIAN_POINT('Ctrl Pts',(-18.1315075132682,21.2417676616992,
-0.147727409065961));
#111475=CARTESIAN_POINT('Ctrl Pts',(-18.0623022558515,21.2186132945629,
-0.152116828781989));
#111476=CARTESIAN_POINT('Ctrl Pts',(-17.9931750162608,21.1954850302612,
-0.156501300131427));
#111477=CARTESIAN_POINT('Ctrl Pts',(-17.9251691345195,21.168757363137,-0.160885771480865));
#111478=CARTESIAN_POINT('Ctrl Pts',(-17.8586810464526,21.138564714753,-0.165270242830304));
#111479=CARTESIAN_POINT('Ctrl Pts',(-17.7922332423914,21.1083903595828,
-0.16965205770286));
#111480=CARTESIAN_POINT('Ctrl Pts',(-17.727301843592,21.0747553873415,-0.174033872575416));
#111481=CARTESIAN_POINT('Ctrl Pts',(-17.6642640090407,21.0378426066978,
-0.178415687447972));
#111482=CARTESIAN_POINT('Ctrl Pts',(-17.6012437811929,21.0009401359321,
-0.182796278463204));
#111483=CARTESIAN_POINT('Ctrl Pts',(-17.5401164818006,20.960761917242,-0.187176869478435));
#111484=CARTESIAN_POINT('Ctrl Pts',(-17.4812338530685,20.9175362525016,
-0.191557460493667));
#111485=CARTESIAN_POINT('Ctrl Pts',(-17.4223484413193,20.8743085447519,
-0.195938258552297));
#111486=CARTESIAN_POINT('Ctrl Pts',(-17.3657082969836,20.8280333908517,
-0.200319056610927));
#111487=CARTESIAN_POINT('Ctrl Pts',(-17.3116340465776,20.7789808973788,
-0.204699854669557));
#111488=CARTESIAN_POINT('Ctrl Pts',(-17.2575026772118,20.7298765894584,
-0.20908528019184));
#111489=CARTESIAN_POINT('Ctrl Pts',(-17.205942969612,20.6779894082539,-0.213470705714123));
#111490=CARTESIAN_POINT('Ctrl Pts',(-17.1572398491782,20.6236274904518,
-0.217856131236407));
#111491=CARTESIAN_POINT('Ctrl Pts',(-17.1085094838157,20.5692351621432,
-0.222244010002017));
#111492=CARTESIAN_POINT('Ctrl Pts',(-17.0626391892087,20.5123657149588,
-0.226631888767627));
#111493=CARTESIAN_POINT('Ctrl Pts',(-17.0198728898629,20.4533595495238,
-0.231019767533237));
#111494=CARTESIAN_POINT('Ctrl Pts',(-16.977030854158,20.3942488879739,-0.235415416949259));
#111495=CARTESIAN_POINT('Ctrl Pts',(-16.9373040526506,20.3329943550554,
-0.239811066365281));
#111496=CARTESIAN_POINT('Ctrl Pts',(-16.9008921528455,20.2699639373939,
-0.244206715781303));
#111497=CARTESIAN_POINT('Ctrl Pts',(-16.876785868281,20.2282350193066,-0.247116829679114));
#111498=CARTESIAN_POINT('Ctrl Pts',(-16.8541315650652,20.1857282478032,
-0.250026943576926));
#111499=CARTESIAN_POINT('Ctrl Pts',(-16.8329755574333,20.1425551882545,
-0.252937057474737));
#111500=CARTESIAN_POINT('Ctrl Pts',(-16.8011149178839,20.0775371889959,
-0.257319646645567));
#111501=CARTESIAN_POINT('Ctrl Pts',(-16.7725299917263,20.0107527148536,
-0.261702235816397));
#111502=CARTESIAN_POINT('Ctrl Pts',(-16.7474198406578,19.9425656296656,
-0.266084824987227));
#111503=CARTESIAN_POINT('Ctrl Pts',(-16.7223474688912,19.8744811348786,
-0.27046082036424));
#111504=CARTESIAN_POINT('Ctrl Pts',(-16.7007396607462,19.804998667962,-0.274836815741254));
#111505=CARTESIAN_POINT('Ctrl Pts',(-16.6827487993224,19.7345050254952,
-0.279212811118268));
#111506=CARTESIAN_POINT('Ctrl Pts',(-16.6647794915184,19.664095836637,-0.283583563914705));
#111507=CARTESIAN_POINT('Ctrl Pts',(-16.6504186420449,19.5926783449243,
-0.287954316711142));
#111508=CARTESIAN_POINT('Ctrl Pts',(-16.6397693071744,19.5206559465391,
-0.292325069507579));
#111509=CARTESIAN_POINT('Ctrl Pts',(-16.6291268685744,19.4486801882446,
-0.296692991902482));
#111510=CARTESIAN_POINT('Ctrl Pts',(-16.6221912467961,19.3761007777963,
-0.301060914297385));
#111511=CARTESIAN_POINT('Ctrl Pts',(-16.6190144407725,19.3033313828498,
-0.305428836692288));
#111512=CARTESIAN_POINT('Ctrl Pts',(-16.6158386365901,19.2305849365467,
-0.309795381613959));
#111513=CARTESIAN_POINT('Ctrl Pts',(-16.6164193161497,19.1576491077123,
-0.314161926535629));
#111514=CARTESIAN_POINT('Ctrl Pts',(-16.6207564869952,19.0849410663896,
-0.3185284714573));
#111515=CARTESIAN_POINT('Ctrl Pts',(-16.6250937309155,19.0122318000445,
-0.322895089948766));
#111516=CARTESIAN_POINT('Ctrl Pts',(-16.6331875609615,18.9397508116576,
-0.327261708440232));
#111517=CARTESIAN_POINT('Ctrl Pts',(-16.6449859783168,18.8679119395679,
-0.331628326931697));
#111518=CARTESIAN_POINT('Ctrl Pts',(-16.6567966078099,18.7959987095216,
-0.335999465160445));
#111519=CARTESIAN_POINT('Ctrl Pts',(-16.6723194019262,18.724729401209,-0.340370603389193));
#111520=CARTESIAN_POINT('Ctrl Pts',(-16.6914510303897,18.65450857442,-0.344741741617941));
#111521=CARTESIAN_POINT('Ctrl Pts',(-16.7105930357156,18.5842496603425,
-0.349115250721693));
#111522=CARTESIAN_POINT('Ctrl Pts',(-16.7333476210311,18.5150408198692,
-0.353488759825446));
#111523=CARTESIAN_POINT('Ctrl Pts',(-16.7595620940047,18.4472697103238,
-0.357862268929199));
#111524=CARTESIAN_POINT('Ctrl Pts',(-16.7858233028864,18.3793777765166,
-0.362243575249389));
#111525=CARTESIAN_POINT('Ctrl Pts',(-16.8155565194802,18.3129291342218,
-0.36662488156958));
#111526=CARTESIAN_POINT('Ctrl Pts',(-16.8485618556778,18.24828924181,-0.37100618788977));
#111527=CARTESIAN_POINT('Ctrl Pts',(-16.8714293819245,18.2035039250521,
-0.374041746645237));
#111528=CARTESIAN_POINT('Ctrl Pts',(-16.895866654182,18.1595863577281,-0.377077305400704));
#111529=CARTESIAN_POINT('Ctrl Pts',(-16.9217951530525,18.1166496937908,
-0.380112864156171));
#111530=CARTESIAN_POINT('Ctrl Pts',(-16.9592870771133,18.0545644125798,
-0.384502201884909));
#111531=CARTESIAN_POINT('Ctrl Pts',(-17.000046146169,17.9942872611044,-0.388891539613648));
#111532=CARTESIAN_POINT('Ctrl Pts',(-17.043872573219,17.9361830401024,-0.393280877342386));
#111533=CARTESIAN_POINT('Ctrl Pts',(-17.0876340137246,17.8781649769917,
-0.397663706489194));
#111534=CARTESIAN_POINT('Ctrl Pts',(-17.1344534950993,17.8223138297408,
-0.402046535636003));
#111535=CARTESIAN_POINT('Ctrl Pts',(-17.1840867641359,17.7689674201693,
-0.406429364782811));
#111536=CARTESIAN_POINT('Ctrl Pts',(-17.2336617334564,17.7156836718046,
-0.410807045816267));
#111537=CARTESIAN_POINT('Ctrl Pts',(-17.2860435979521,17.6648991677451,
-0.415184726849724));
#111538=CARTESIAN_POINT('Ctrl Pts',(-17.3409475304282,17.6169191309661,
-0.41956240788318));
#111539=CARTESIAN_POINT('Ctrl Pts',(-17.3958166506481,17.5689695162945,
-0.423937313214652));
#111540=CARTESIAN_POINT('Ctrl Pts',(-17.4532043037707,17.5238211571202,
-0.428312218546124));
#111541=CARTESIAN_POINT('Ctrl Pts',(-17.512789475476,17.4817418195099,-0.432687123877597));
#111542=CARTESIAN_POINT('Ctrl Pts',(-17.5723564947757,17.4396753012167,
-0.437060696410096));
#111543=CARTESIAN_POINT('Ctrl Pts',(-17.6341193099784,17.4006762261877,
-0.441434268942594));
#111544=CARTESIAN_POINT('Ctrl Pts',(-17.697725898141,17.3649704807842,-0.445807841475093));
#111545=CARTESIAN_POINT('Ctrl Pts',(-17.7613340609316,17.3292638514586,
-0.450181522278611));
#111546=CARTESIAN_POINT('Ctrl Pts',(-17.8267856659411,17.29685094787,-0.454555203082129));
#111547=CARTESIAN_POINT('Ctrl Pts',(-17.8937034068912,17.2679120875242,
-0.458928883885646));
#111548=CARTESIAN_POINT('Ctrl Pts',(-17.9606903750841,17.2389432895641,
-0.463307089316843));
#111549=CARTESIAN_POINT('Ctrl Pts',(-18.0291460640641,17.2134559021899,
-0.46768529474804));
#111550=CARTESIAN_POINT('Ctrl Pts',(-18.0986732370017,17.1915820382551,
-0.472063500179237));
#111551=CARTESIAN_POINT('Ctrl Pts',(-18.1682382801081,17.1696962600299,
-0.476444090338188));
#111552=CARTESIAN_POINT('Ctrl Pts',(-18.2388755021191,17.1514280448653,
-0.480824680497139));
#111553=CARTESIAN_POINT('Ctrl Pts',(-18.3101751880181,17.1368588455102,
-0.48520527065609));
#111554=CARTESIAN_POINT('Ctrl Pts',(-18.3816008664645,17.1222639011532,
-0.489593601686642));
#111555=CARTESIAN_POINT('Ctrl Pts',(-18.4536908693965,17.1113810977932,
-0.493981932717193));
#111556=CARTESIAN_POINT('Ctrl Pts',(-18.5260286230796,17.1042401877808,
-0.498370263747745));
#111557=CARTESIAN_POINT('Ctrl Pts',(-18.5750326393233,17.0994026962577,
-0.501343066111032));
#111558=CARTESIAN_POINT('Ctrl Pts',(-18.624150260615,17.0962813311373,-0.504315868474319));
#111559=CARTESIAN_POINT('Ctrl Pts',(-18.6732524681258,17.0948717578154,
-0.507288670837606));
#111560=CARTESIAN_POINT('Ctrl Pts',(-18.7457477325719,17.0927906417942,
-0.511677762579042));
#111561=CARTESIAN_POINT('Ctrl Pts',(-18.818490899314,17.0944351534906,-0.516066854320478));
#111562=CARTESIAN_POINT('Ctrl Pts',(-18.8910671105736,17.0998347002719,
-0.520455946061914));
#111563=CARTESIAN_POINT('Ctrl Pts',(-18.9635359557306,17.1052262591976,
-0.524838544771178));
#111564=CARTESIAN_POINT('Ctrl Pts',(-19.035837858837,17.1143617900503,-0.529221143480442));
#111565=CARTESIAN_POINT('Ctrl Pts',(-19.1075565880863,17.1272187073742,
-0.533603742189706));
#111566=CARTESIAN_POINT('Ctrl Pts',(-19.1791914726444,17.1400605939763,
-0.537981217305189));
#111567=CARTESIAN_POINT('Ctrl Pts',(-19.2502440654555,17.1566151398615,
-0.542358692420672));
#111568=CARTESIAN_POINT('Ctrl Pts',(-19.320303591177,17.1768079984984,-0.546736167536156));
#111569=CARTESIAN_POINT('Ctrl Pts',(-19.3903189366748,17.1969881233207,
-0.55111088217292));
#111570=CARTESIAN_POINT('Ctrl Pts',(-19.4593419954755,17.2208018753163,
-0.555485596809685));
#111571=CARTESIAN_POINT('Ctrl Pts',(-19.5269739113634,17.2481242077255,
-0.55986031144645));
#111572=CARTESIAN_POINT('Ctrl Pts',(-19.5945854628885,17.2754383132218,
-0.564233708831224));
#111573=CARTESIAN_POINT('Ctrl Pts',(-19.6608062563393,17.3062587212117,
-0.568607106215997));
#111574=CARTESIAN_POINT('Ctrl Pts',(-19.725255876789,17.3404116469059,-0.572980503600771));
#111575=CARTESIAN_POINT('Ctrl Pts',(-19.7897073269138,17.3745655421753,
-0.577354025142924));
#111576=CARTESIAN_POINT('Ctrl Pts',(-19.8523870791116,17.4120519154598,
-0.581727546685077));
#111577=CARTESIAN_POINT('Ctrl Pts',(-19.9129393606857,17.4526510631203,
-0.58610106822723));
#111578=CARTESIAN_POINT('Ctrl Pts',(-19.973554643469,17.4932924518876,-0.590479140170093));
#111579=CARTESIAN_POINT('Ctrl Pts',(-20.0320376349008,17.5370528121332,
-0.594857212112955));
#111580=CARTESIAN_POINT('Ctrl Pts',(-20.0880623158587,17.5836695956963,
-0.599235284055817));
#111581=CARTESIAN_POINT('Ctrl Pts',(-20.1441176953746,17.6303119227879,
-0.60361575495024));
#111582=CARTESIAN_POINT('Ctrl Pts',(-20.1977117280629,17.6798134620823,
-0.607996225844662));
#111583=CARTESIAN_POINT('Ctrl Pts',(-20.2485542488445,17.731873762214,-0.612376696739084));
#111584=CARTESIAN_POINT('Ctrl Pts',(-20.2994868988124,17.7840263503049,
-0.616764932950229));
#111585=CARTESIAN_POINT('Ctrl Pts',(-20.3476579775569,17.8387463951233,
-0.621153169161374));
#111586=CARTESIAN_POINT('Ctrl Pts',(-20.392817087906,17.8956997039189,-0.625541405372519));
#111587=CARTESIAN_POINT('Ctrl Pts',(-20.4234260448481,17.9343027978054,
-0.628515762754692));
#111588=CARTESIAN_POINT('Ctrl Pts',(-20.4526521208593,17.9739312228937,
-0.631490120136865));
#111589=CARTESIAN_POINT('Ctrl Pts',(-20.4804290546179,18.0144739630136,
-0.634464477519039));
#111590=CARTESIAN_POINT('Ctrl Pts',(-20.5219934548532,18.0751406547235,
-0.638915198457137));
#111591=CARTESIAN_POINT('Ctrl Pts',(-20.5604706098725,18.1380885636268,
-0.643365919395235));
#111592=CARTESIAN_POINT('Ctrl Pts',(-20.5956058248693,18.2029758173473,
-0.647816640333333));
#111593=CARTESIAN_POINT('Ctrl Pts',(-20.630675943178,18.2677428513588,-0.652259115208526));
#111594=CARTESIAN_POINT('Ctrl Pts',(-20.6624162095655,18.3344416830545,
-0.656701590083719));
#111595=CARTESIAN_POINT('Ctrl Pts',(-20.6906150240255,18.4027013870123,
-0.661144064958911));
#111596=CARTESIAN_POINT('Ctrl Pts',(-20.7018340891964,18.4298589140898,
-0.662911529871862));
#111597=CARTESIAN_POINT('Ctrl Pts',(-20.7124930667491,18.4572631970918,
-0.664678994784814));
#111598=CARTESIAN_POINT('Ctrl Pts',(-20.7225806137986,18.4848897174502,
-0.666446459697765));
#111599=CARTESIAN_POINT('Origin',(-18.734,19.211,0.));
#111600=CARTESIAN_POINT('',(-20.8509997094738,19.2121090932814,-0.710943720977507));
#111601=CARTESIAN_POINT('Ctrl Pts',(-20.7225806137986,18.4848897174502,
-0.666446459697765));
#111602=CARTESIAN_POINT('Ctrl Pts',(-20.7478890253796,18.5542012502099,
-0.6708808112059));
#111603=CARTESIAN_POINT('Ctrl Pts',(-20.7695972005712,18.6249130163545,
-0.675315162714036));
#111604=CARTESIAN_POINT('Ctrl Pts',(-20.7875591148731,18.696622743775,-0.679749514222171));
#111605=CARTESIAN_POINT('Ctrl Pts',(-20.8055066444181,18.7682750426286,
-0.684180314490311));
#111606=CARTESIAN_POINT('Ctrl Pts',(-20.819713760552,18.8409232657494,-0.688611114758451));
#111607=CARTESIAN_POINT('Ctrl Pts',(-20.8300842049517,18.914149859774,-0.69304191502659));
#111608=CARTESIAN_POINT('Ctrl Pts',(-20.8404495516885,18.987340458766,-0.697470537304587));
#111609=CARTESIAN_POINT('Ctrl Pts',(-20.8469819094182,19.0611084042472,
-0.701899159582584));
#111610=CARTESIAN_POINT('Ctrl Pts',(-20.8496363438536,19.135027238001,-0.70632778186058));
#111611=CARTESIAN_POINT('Ctrl Pts',(-20.8505585800838,19.1607090275647,
-0.707866428232889));
#111612=CARTESIAN_POINT('Ctrl Pts',(-20.8510131737292,19.1864089784392,
-0.709405074605198));
#111613=CARTESIAN_POINT('Ctrl Pts',(-20.8509997094738,19.2121090932814,
-0.710943720977507));
#111614=CARTESIAN_POINT('Ctrl Pts',(-20.8509997571974,19.2120139161396,
-0.712619133284185));
#111615=CARTESIAN_POINT('Ctrl Pts',(-20.8509644874188,19.2856552261446,
-0.716802597200607));
#111616=CARTESIAN_POINT('Ctrl Pts',(-20.847086770126,19.3592496595573,-0.720880559931813));
#111617=CARTESIAN_POINT('Ctrl Pts',(-20.8222620020048,19.595214125847,-0.733864837499567));
#111618=CARTESIAN_POINT('Ctrl Pts',(-20.7863401949605,19.7553767871956,
-0.742508191233821));
#111619=CARTESIAN_POINT('Ctrl Pts',(-20.7220379866568,19.9392645428959,
-0.753708987400108));
#111620=CARTESIAN_POINT('Ctrl Pts',(-20.7110792378879,19.9685102205914,
-0.75553220632609));
#111621=CARTESIAN_POINT('Ctrl Pts',(-20.6968237939304,20.0041347978913,
-0.757817282440839));
#111622=CARTESIAN_POINT('Ctrl Pts',(-20.6941357135984,20.0107549841072,
-0.758244682239247));
#111623=CARTESIAN_POINT('Ctrl Pts',(-20.6898577693182,20.0211395457907,
-0.758919647536638));
#111624=CARTESIAN_POINT('Ctrl Pts',(-20.6882904028546,20.0249132128897,
-0.759165870600361));
#111625=CARTESIAN_POINT('Ctrl Pts',(-20.6853317611769,20.0319787634579,
-0.75962869952792));
#111626=CARTESIAN_POINT('Ctrl Pts',(-20.6839430718721,20.0352716712264,
-0.759845148210268));
#111627=CARTESIAN_POINT('Ctrl Pts',(-20.6807434917007,20.042805290023,-0.760342046420319));
#111628=CARTESIAN_POINT('Ctrl Pts',(-20.6789270824204,20.0470436030065,
-0.760622828751681));
#111629=CARTESIAN_POINT('Ctrl Pts',(-20.6732663761397,20.0601337089901,
-0.761493774946246));
#111630=CARTESIAN_POINT('Ctrl Pts',(-20.6693754502033,20.0689650296054,
-0.762086675123137));
#111631=CARTESIAN_POINT('Ctrl Pts',(-20.6287967220064,20.1593867246904,
-0.768209612911351));
#111632=CARTESIAN_POINT('Ctrl Pts',(-20.5870364700279,20.2385914074892,
-0.7740093348254));
#111633=CARTESIAN_POINT('Ctrl Pts',(-20.4754719849046,20.4211519047305,
-0.788069021307969));
#111634=CARTESIAN_POINT('Ctrl Pts',(-20.4012933161308,20.5214689210608,
-0.796363873212959));
#111635=CARTESIAN_POINT('Ctrl Pts',(-20.276280420012,20.6626053145,-0.808564248865147));
#111636=CARTESIAN_POINT('Ctrl Pts',(-20.2316806753148,20.708578286057,-0.812641832944686));
#111637=CARTESIAN_POINT('Ctrl Pts',(-20.1666557738227,20.7697897404679,
-0.818210628129412));
#111638=CARTESIAN_POINT('Ctrl Pts',(-20.147939876371,20.7867861952464,-0.819773459131753));
#111639=CARTESIAN_POINT('Ctrl Pts',(-20.1190927133919,20.8120552684204,
-0.822123071126478));
#111640=CARTESIAN_POINT('Ctrl Pts',(-20.1091823322634,20.820575522391,-0.822920016855451));
#111641=CARTESIAN_POINT('Ctrl Pts',(-20.0907767487775,20.8361052671643,
-0.824381527496059));
#111642=CARTESIAN_POINT('Ctrl Pts',(-20.0823045815443,20.8431412432604,
-0.825047164872525));
#111643=CARTESIAN_POINT('Ctrl Pts',(-20.0684848163721,20.8544372539313,
-0.826121634120932));
#111644=CARTESIAN_POINT('Ctrl Pts',(-20.0631708905226,20.8587379883434,
-0.82653211244437));
#111645=CARTESIAN_POINT('Ctrl Pts',(-20.0528357104379,20.8670200573879,
-0.827325344376364));
#111646=CARTESIAN_POINT('Ctrl Pts',(-20.0478170344389,20.871004476804,-0.827708219487189));
#111647=CARTESIAN_POINT('Ctrl Pts',(-20.0362987645331,20.8800640874097,
-0.82858172565631));
#111648=CARTESIAN_POINT('Ctrl Pts',(-20.0297874270979,20.885124232755,-0.829071754163217));
#111649=CARTESIAN_POINT('Ctrl Pts',(-20.0127186575559,20.8982296149092,
-0.830346638840626));
#111650=CARTESIAN_POINT('Ctrl Pts',(-20.0021147343949,20.9062139130508,
-0.831129096273738));
#111651=CARTESIAN_POINT('Ctrl Pts',(-19.9282389158269,20.9607581179443,
-0.83651618177468));
#111652=CARTESIAN_POINT('Ctrl Pts',(-19.8624894643728,21.003867420594,-0.840984804573554));
#111653=CARTESIAN_POINT('Ctrl Pts',(-19.6590188628693,21.1216359093979,
-0.854082781571101));
#111654=CARTESIAN_POINT('Ctrl Pts',(-19.5152783900345,21.1847757490113,
-0.862369425581119));
#111655=CARTESIAN_POINT('Ctrl Pts',(-19.3162813833807,21.2470107542544,
-0.873917128287804));
#111656=CARTESIAN_POINT('Ctrl Pts',(-19.2661150801762,21.2606936873164,
-0.876838311748348));
#111657=CARTESIAN_POINT('Ctrl Pts',(-19.188878892102,21.2787334268187,-0.881419646854493));
#111658=CARTESIAN_POINT('Ctrl Pts',(-19.1621414977169,21.2844345971685,
-0.883020721231884));
#111659=CARTESIAN_POINT('Ctrl Pts',(-19.1285733413727,21.2909153468698,
-0.885058118865585));
#111660=CARTESIAN_POINT('Ctrl Pts',(-19.1218378389243,21.2921818228192,
-0.885468292525569));
#111661=CARTESIAN_POINT('Ctrl Pts',(-19.1111362675934,21.294140284196,-0.886122326229782));
#111662=CARTESIAN_POINT('Ctrl Pts',(-19.1071741028785,21.2948537127864,
-0.886364984222708));
#111663=CARTESIAN_POINT('Ctrl Pts',(-19.099675739095,21.2961817993719,-0.886825213188938));
#111664=CARTESIAN_POINT('Ctrl Pts',(-19.0961400036328,21.2967987677715,
-0.887042651213709));
#111665=CARTESIAN_POINT('Ctrl Pts',(-19.0880231761644,21.2981938536432,
-0.887542773090114));
#111666=CARTESIAN_POINT('Ctrl Pts',(-19.0834410843493,21.2989658808437,
-0.887825798261902));
#111667=CARTESIAN_POINT('Ctrl Pts',(-19.071206252694,21.3009859007711,-0.888583307904103));
#111668=CARTESIAN_POINT('Ctrl Pts',(-19.0635492186102,21.3022069315537,
-0.889059256198721));
#111669=CARTESIAN_POINT('Ctrl Pts',(-19.0080358175804,21.3107469313232,
-0.892522552686661));
#111670=CARTESIAN_POINT('Ctrl Pts',(-18.9599513418803,21.3164638435916,
-0.895590319796249));
#111671=CARTESIAN_POINT('Ctrl Pts',(-18.9040180682394,21.3211759547509,
-0.899205847696877));
#111672=CARTESIAN_POINT('Ctrl Pts',(-18.896315118878,21.3217824386576,-0.899704802798105));
#111673=CARTESIAN_POINT('Ctrl Pts',(-18.7362031820373,21.3335070701645,
-0.910095381370922));
#111674=CARTESIAN_POINT('Ctrl Pts',(-18.5830358157563,21.3281335954217,
-0.920358116998048));
#111675=CARTESIAN_POINT('Ctrl Pts',(-18.3399050110413,21.2930647988216,
-0.936301292287723));
#111676=CARTESIAN_POINT('Ctrl Pts',(-18.2489969350588,21.2737846834032,
-0.942191496674143));
#111677=CARTESIAN_POINT('Ctrl Pts',(-18.1393445762057,21.242875597218,-0.949187253272218));
#111678=CARTESIAN_POINT('Ctrl Pts',(-18.119137872333,21.2368524452801,-0.950472112144795));
#111679=CARTESIAN_POINT('Ctrl Pts',(-18.0904786757538,21.227841477502,-0.952288825887074));
#111680=CARTESIAN_POINT('Ctrl Pts',(-18.0819504618521,21.2251004552375,
-0.952828721196307));
#111681=CARTESIAN_POINT('Ctrl Pts',(-18.0672480883332,21.2202718483831,
-0.953758328574996));
#111682=CARTESIAN_POINT('Ctrl Pts',(-18.0610657480937,21.2182097465142,
-0.954148873460335));
#111683=CARTESIAN_POINT('Ctrl Pts',(-18.0492328464613,21.2142021009902,
-0.954895725948036));
#111684=CARTESIAN_POINT('Ctrl Pts',(-18.0435808167235,21.2122611185121,
-0.955252179838339));
#111685=CARTESIAN_POINT('Ctrl Pts',(-18.0288748718741,21.2071411850671,
-0.956178936265384));
#111686=CARTESIAN_POINT('Ctrl Pts',(-18.0198341521834,21.2039245403315,
-0.956747984307098));
#111687=CARTESIAN_POINT('Ctrl Pts',(-17.9889263123131,21.1926903483604,
-0.958691292278482));
#111688=CARTESIAN_POINT('Ctrl Pts',(-17.9671693056927,21.1843733013344,
-0.960055577346037));
#111689=CARTESIAN_POINT('Ctrl Pts',(-17.7867477354959,21.1119689216963,
-0.971348978071564));
#111690=CARTESIAN_POINT('Ctrl Pts',(-17.6362548081601,21.0292222243391,
-0.980569978519324));
#111691=CARTESIAN_POINT('Ctrl Pts',(-17.4241948340607,20.8766001513782,
-0.994776638331962));
#111692=CARTESIAN_POINT('Ctrl Pts',(-17.3544796360186,20.8193328079773,
-0.999701344985896));
#111693=CARTESIAN_POINT('Ctrl Pts',(-17.2604243215597,20.7314453644377,
-1.00704506081657));
#111694=CARTESIAN_POINT('Ctrl Pts',(-17.2329451248067,20.7043228804672,
-1.00928622953275));
#111695=CARTESIAN_POINT('Ctrl Pts',(-17.2009530100053,20.670970520954,-1.01203567414906));
#111696=CARTESIAN_POINT('Ctrl Pts',(-17.1957110727717,20.665446344133,-1.01249086182849));
#111697=CARTESIAN_POINT('Ctrl Pts',(-17.1876303834867,20.6568380194722,
-1.01320009247586));
#111698=CARTESIAN_POINT('Ctrl Pts',(-17.1847707323466,20.6537734558738,
-1.01345256142014));
#111699=CARTESIAN_POINT('Ctrl Pts',(-17.1794973944048,20.6480884947147,
-1.01392092107518));
#111700=CARTESIAN_POINT('Ctrl Pts',(-17.1770812137249,20.6454704893504,
-1.01413661643034));
#111701=CARTESIAN_POINT('Ctrl Pts',(-17.1716502496337,20.6395559888072,
-1.01462392428141));
#111702=CARTESIAN_POINT('Ctrl Pts',(-17.1686393037645,20.6362560631204,
-1.01489581947224));
#111703=CARTESIAN_POINT('Ctrl Pts',(-17.1598306450122,20.6265403976705,
-1.01569629081882));
#111704=CARTESIAN_POINT('Ctrl Pts',(-17.1540618521074,20.6200987256406,
-1.01622696190097));
#111705=CARTESIAN_POINT('Ctrl Pts',(-17.1140894207959,20.5749098063458,
-1.01994813811215));
#111706=CARTESIAN_POINT('Ctrl Pts',(-17.081278129716,20.5349598601349,-1.02322979657745));
#111707=CARTESIAN_POINT('Ctrl Pts',(-17.036605646116,20.476317108393,-1.02798904859693));
#111708=CARTESIAN_POINT('Ctrl Pts',(-17.0235219917822,20.4585736105255,
-1.02942192098114));
#111709=CARTESIAN_POINT('Ctrl Pts',(-16.9840406604591,20.4032419330316,
-1.03386143163218));
#111710=CARTESIAN_POINT('Ctrl Pts',(-16.958587554632,20.3649969545664,-1.03688966893136));
#111711=CARTESIAN_POINT('Ctrl Pts',(-16.8768044647256,20.2329944378632,
-1.0471474763071));
#111712=CARTESIAN_POINT('Ctrl Pts',(-16.8264950004093,20.1357032123579,
-1.05437846374188));
#111713=CARTESIAN_POINT('Ctrl Pts',(-16.7624917997307,19.984225277447,-1.06494833635042));
#111714=CARTESIAN_POINT('Ctrl Pts',(-16.7430437086544,19.9326756746082,
-1.06843562985732));
#111715=CARTESIAN_POINT('Ctrl Pts',(-16.7147841280757,19.8478924823877,
-1.07399054196894));
#111716=CARTESIAN_POINT('Ctrl Pts',(-16.704732821792,19.8151023978544,-1.07609656105327));
#111717=CARTESIAN_POINT('Ctrl Pts',(-16.6925670134059,19.7716756027844,
-1.07883211206632));
#111718=CARTESIAN_POINT('Ctrl Pts',(-16.6897316546778,19.761247861793,-1.07948496914327));
#111719=CARTESIAN_POINT('Ctrl Pts',(-16.6852176273085,19.7441297747803,
-1.08055025475023));
#111720=CARTESIAN_POINT('Ctrl Pts',(-16.6834916170951,19.7374522208109,
-1.08096421211433));
#111721=CARTESIAN_POINT('Ctrl Pts',(-16.680213173264,19.7245078873784,-1.08176361527494));
#111722=CARTESIAN_POINT('Ctrl Pts',(-16.6786567155513,19.7182422148946,
-1.08214918730627));
#111723=CARTESIAN_POINT('Ctrl Pts',(-16.6751283415835,19.7037554830237,
-1.08303752944692));
#111724=CARTESIAN_POINT('Ctrl Pts',(-16.6731769512605,19.6955295004719,
-1.08353963339714));
#111725=CARTESIAN_POINT('Ctrl Pts',(-16.6680598863212,19.6733685164413,
-1.08488620753554));
#111726=CARTESIAN_POINT('Ctrl Pts',(-16.664985905864,19.659412635284,-1.08572773572183));
#111727=CARTESIAN_POINT('Ctrl Pts',(-16.6380608209679,19.5309965610869,
-1.09341431787822));
#111728=CARTESIAN_POINT('Ctrl Pts',(-16.6235871599688,19.4147688836979,
-1.09994216807236));
#111729=CARTESIAN_POINT('Ctrl Pts',(-16.6120973758036,19.1351849122773,
-1.11526010212648));
#111730=CARTESIAN_POINT('Ctrl Pts',(-16.6242137323605,18.972235145299,-1.12386691866123));
#111731=CARTESIAN_POINT('Ctrl Pts',(-16.6609680655026,18.7805676774271,
-1.13507496762888));
#111732=CARTESIAN_POINT('Ctrl Pts',(-16.6677798930822,18.7489744611762,
-1.13696011689814));
#111733=CARTESIAN_POINT('Ctrl Pts',(-16.6769959440115,18.7105246992441,
-1.13931436159752));
#111734=CARTESIAN_POINT('Ctrl Pts',(-16.6787161466169,18.7035066585481,
-1.13974653461169));
#111735=CARTESIAN_POINT('Ctrl Pts',(-16.6814701959169,18.6925144501394,
-1.14042750463657));
#111736=CARTESIAN_POINT('Ctrl Pts',(-16.6824797534705,18.6885341738594,
-1.14067492227184));
#111737=CARTESIAN_POINT('Ctrl Pts',(-16.6843891984449,18.6810968739097,
-1.14113884384032));
#111738=CARTESIAN_POINT('Ctrl Pts',(-16.6852862576736,18.6776391819487,
-1.14135518358945));
#111739=CARTESIAN_POINT('Ctrl Pts',(-16.6873549154763,18.6697478147095,
-1.14185041999644));
#111740=CARTESIAN_POINT('Ctrl Pts',(-16.6885321679357,18.6653156799367,
-1.14212964011229));
#111741=CARTESIAN_POINT('Ctrl Pts',(-16.6921981560382,18.6516924817732,
-1.14299111899549));
#111742=CARTESIAN_POINT('Ctrl Pts',(-16.6947344695324,18.6425145046581,
-1.14357603093432));
#111743=CARTESIAN_POINT('Ctrl Pts',(-16.7185345291006,18.5586001020669,
-1.1489634870136));
#111744=CARTESIAN_POINT('Ctrl Pts',(-16.743833883568,18.4850779475505,-1.15397035239638));
#111745=CARTESIAN_POINT('Ctrl Pts',(-16.7885262290105,18.3752408746039,
-1.16173151612132));
#111746=CARTESIAN_POINT('Ctrl Pts',(-16.8050338382097,18.3378156385795,
-1.16442854162162));
#111747=CARTESIAN_POINT('Ctrl Pts',(-16.8696062210673,18.2022022690548,
-1.17435060277607));
#111748=CARTESIAN_POINT('Ctrl Pts',(-16.9241744305047,18.1072917502362,
-1.18157790916052));
#111749=CARTESIAN_POINT('Ctrl Pts',(-17.0168586192068,17.9715885596055,
-1.19214010318181));
#111750=CARTESIAN_POINT('Ctrl Pts',(-17.0496456235718,17.9273854191799,
-1.19562339839137));
#111751=CARTESIAN_POINT('Ctrl Pts',(-17.1055890508072,17.8578034999957,
-1.20117279033525));
#111752=CARTESIAN_POINT('Ctrl Pts',(-17.1277042788828,17.8316243227604,
-1.20327718171052));
#111753=CARTESIAN_POINT('Ctrl Pts',(-17.1576168939423,17.7979104643993,
-1.20601104221214));
#111754=CARTESIAN_POINT('Ctrl Pts',(-17.1648493365256,17.7898835604415,
-1.206663793652));
#111755=CARTESIAN_POINT('Ctrl Pts',(-17.1767991192414,17.7768235844802,
-1.20772900343561));
#111756=CARTESIAN_POINT('Ctrl Pts',(-17.1814801023337,17.7717576496746,
-1.20814298933927));
#111757=CARTESIAN_POINT('Ctrl Pts',(-17.190591363699,17.7619932775971,-1.20894251483392));
#111758=CARTESIAN_POINT('Ctrl Pts',(-17.1950185401579,17.7572920623917,
-1.20932818032899));
#111759=CARTESIAN_POINT('Ctrl Pts',(-17.2052937035856,17.7464804224071,
-1.21021683459015));
#111760=CARTESIAN_POINT('Ctrl Pts',(-17.2111569614164,17.7403846128733,
-1.21071915639667));
#111761=CARTESIAN_POINT('Ctrl Pts',(-17.2270311478431,17.7240775543239,
-1.21206653225809));
#111762=CARTESIAN_POINT('Ctrl Pts',(-17.2371093742525,17.713932215858,-1.21290864003686));
#111763=CARTESIAN_POINT('Ctrl Pts',(-17.3310033182662,17.6213092191099,
-1.22063513862648));
#111764=CARTESIAN_POINT('Ctrl Pts',(-17.4214564833862,17.5458419534176,
-1.22719844412912));
#111765=CARTESIAN_POINT('Ctrl Pts',(-17.6516587521603,17.3842528929774,
-1.24259191487288));
#111766=CARTESIAN_POINT('Ctrl Pts',(-17.7960287792519,17.3060944366576,
-1.25123873227028));
#111767=CARTESIAN_POINT('Ctrl Pts',(-17.9767198091943,17.2338362009708,
-1.26243143158562));
#111768=CARTESIAN_POINT('Ctrl Pts',(-18.0057508762016,17.2229600203372,
-1.26424162530969));
#111769=CARTESIAN_POINT('Ctrl Pts',(-18.0417424947828,17.2103702386494,
-1.26651246501864));
#111770=CARTESIAN_POINT('Ctrl Pts',(-18.0484882642279,17.2080487893232,
-1.26693921807486));
#111771=CARTESIAN_POINT('Ctrl Pts',(-18.0591164756236,17.2044512391706,
-1.2676135606256));
#111772=CARTESIAN_POINT('Ctrl Pts',(-18.0629911707342,17.2031521841886,
-1.26785981548969));
#111773=CARTESIAN_POINT('Ctrl Pts',(-18.0702630935823,17.2007375532514,
-1.26832279388764));
#111774=CARTESIAN_POINT('Ctrl Pts',(-18.0736593943947,17.1996193623134,
-1.26853936072229));
#111775=CARTESIAN_POINT('Ctrl Pts',(-18.0814483277144,17.1970768040885,
-1.2690367849795));
#111776=CARTESIAN_POINT('Ctrl Pts',(-18.0858427856537,17.1956582055167,
-1.26931797660527));
#111777=CARTESIAN_POINT('Ctrl Pts',(-18.0994689238567,17.191308655185,-1.27019150285857));
#111778=CARTESIAN_POINT('Ctrl Pts',(-18.1087159515204,17.1884267218595,
-1.27078659716504));
#111779=CARTESIAN_POINT('Ctrl Pts',(-18.2199199388366,17.154604307949,-1.27796792724048));
#111780=CARTESIAN_POINT('Ctrl Pts',(-18.3240413118227,17.1313437695978,
-1.28493417481822));
#111781=CARTESIAN_POINT('Ctrl Pts',(-18.5377573258039,17.1002762461415,
-1.29918061398552));
#111782=CARTESIAN_POINT('Ctrl Pts',(-18.6471234135829,17.0929534442292,
-1.3064404179305));
#111783=CARTESIAN_POINT('Ctrl Pts',(-18.8191816468751,17.0947878546033,
-1.31756393534099));
#111784=CARTESIAN_POINT('Ctrl Pts',(-18.881737767282,17.0982329799035,-1.32154887540623));
#111785=CARTESIAN_POINT('Ctrl Pts',(-18.968826740589,17.1069170190539,-1.32700390271539));
#111786=CARTESIAN_POINT('Ctrl Pts',(-18.9935547201064,17.1098240868105,
-1.32854246794858));
#111787=CARTESIAN_POINT('Ctrl Pts',(-19.0367600611059,17.1156777949324,
-1.33121312760618));
#111788=CARTESIAN_POINT('Ctrl Pts',(-19.0552599654708,17.1184343815603,
-1.33235100316907));
#111789=CARTESIAN_POINT('Ctrl Pts',(-19.0821458078013,17.1228054824148,
-1.33399684596642));
#111790=CARTESIAN_POINT('Ctrl Pts',(-19.0905619617199,17.1242260741639,
-1.33451092929524));
#111791=CARTESIAN_POINT('Ctrl Pts',(-19.1053191105548,17.1268088686221,
-1.3354104383561));
#111792=CARTESIAN_POINT('Ctrl Pts',(-19.1116637739917,17.1279492014793,
-1.33579655352527));
#111793=CARTESIAN_POINT('Ctrl Pts',(-19.1239855686781,17.1302219573573,
-1.33654525053515));
#111794=CARTESIAN_POINT('Ctrl Pts',(-19.1299632158707,17.1313511980657,
-1.33690792949389));
#111795=CARTESIAN_POINT('Ctrl Pts',(-19.1442608149774,17.1341160459722,
-1.33777416058269));
#111796=CARTESIAN_POINT('Ctrl Pts',(-19.1525760123578,17.1357759109289,
-1.33827693555516));
#111797=CARTESIAN_POINT('Ctrl Pts',(-19.1826607657826,17.141969556595,-1.34009252945942));
#111798=CARTESIAN_POINT('Ctrl Pts',(-19.2043690043141,17.1467963972756,
-1.34139599484094));
#111799=CARTESIAN_POINT('Ctrl Pts',(-19.4052505677662,17.1947961940575,
-1.35340661079202));
#111800=CARTESIAN_POINT('Ctrl Pts',(-19.578138660735,17.2608484261107,-1.36327116938842));
#111801=CARTESIAN_POINT('Ctrl Pts',(-19.8115611527497,17.3869628521163,
-1.3777304877114));
#111802=CARTESIAN_POINT('Ctrl Pts',(-19.8805489176555,17.429519413392,-1.38218222351613));
#111803=CARTESIAN_POINT('Ctrl Pts',(-19.9766417376677,17.4966939345755,
-1.38888709278125));
#111804=CARTESIAN_POINT('Ctrl Pts',(-20.005819439317,17.5182275010892,-1.39099582174232));
#111805=CARTESIAN_POINT('Ctrl Pts',(-20.0403302155074,17.5450929441108,
-1.39359845490154));
#111806=CARTESIAN_POINT('Ctrl Pts',(-20.0462081306796,17.5497189374463,
-1.39404564302806));
#111807=CARTESIAN_POINT('Ctrl Pts',(-20.0553184366203,17.5569673782921,
-1.3947450683031));
#111808=CARTESIAN_POINT('Ctrl Pts',(-20.058567884312,17.5595684259435,-1.39499580052242));
#111809=CARTESIAN_POINT('Ctrl Pts',(-20.0645866224007,17.5644153670785,
-1.39546260918367));
#111810=CARTESIAN_POINT('Ctrl Pts',(-20.0673579172715,17.5666586799171,
-1.39567850094296));
#111811=CARTESIAN_POINT('Ctrl Pts',(-20.0736189729604,17.571753125808,-1.39616840971934));
#111812=CARTESIAN_POINT('Ctrl Pts',(-20.0771052872768,17.5746083923203,
-1.39644272284676));
#111813=CARTESIAN_POINT('Ctrl Pts',(-20.0873944228759,17.5830901522574,
-1.39725674035497));
#111814=CARTESIAN_POINT('Ctrl Pts',(-20.0941710972335,17.5887480108595,
-1.39779864466668));
#111815=CARTESIAN_POINT('Ctrl Pts',(-20.1437891457519,17.630703671618,-1.40180783895269));
#111816=CARTESIAN_POINT('Ctrl Pts',(-20.1852029484385,17.6686476611607,
-1.4053826159621));
#111817=CARTESIAN_POINT('Ctrl Pts',(-20.2694058430704,17.7521918859532,
-1.41306229560888));
#111818=CARTESIAN_POINT('Ctrl Pts',(-20.311784641918,17.7981350999428,-1.41717759412954));
#111819=CARTESIAN_POINT('Ctrl Pts',(-20.4227518524972,17.9296641046729,
-1.42854454226548));
#111820=CARTESIAN_POINT('Ctrl Pts',(-20.4868272563151,18.0188152136544,
-1.43579415293509));
#111821=CARTESIAN_POINT('Ctrl Pts',(-20.5724488815152,18.1598759155566,
-1.44640315108994));
#111822=CARTESIAN_POINT('Ctrl Pts',(-20.5993182114281,18.2083310946217,
-1.44991079691162));
#111823=CARTESIAN_POINT('Ctrl Pts',(-20.6397608263552,18.2885304252743,
-1.45549437506563));
#111824=CARTESIAN_POINT('Ctrl Pts',(-20.6545119656725,18.3196479640476,
-1.45760919717485));
#111825=CARTESIAN_POINT('Ctrl Pts',(-20.6728942765733,18.3610028708258,
-1.46035438236236));
#111826=CARTESIAN_POINT('Ctrl Pts',(-20.677214501923,18.3709264665149,-1.46100827245335));
#111827=CARTESIAN_POINT('Ctrl Pts',(-20.6841645614341,18.3872313378617,
-1.46207484230072));
#111828=CARTESIAN_POINT('Ctrl Pts',(-20.6868395896257,18.3935930240452,
-1.46248905750794));
#111829=CARTESIAN_POINT('Ctrl Pts',(-20.6919565570171,18.4059305668096,
-1.46328868198003));
#111830=CARTESIAN_POINT('Ctrl Pts',(-20.6944023615243,18.4119047279714,
-1.46367421894243));
#111831=CARTESIAN_POINT('Ctrl Pts',(-20.6999852446905,18.4257214744577,
-1.4645620858008));
#111832=CARTESIAN_POINT('Ctrl Pts',(-20.7031028026407,18.4335718677551,
-1.46506375223575));
#111833=CARTESIAN_POINT('Ctrl Pts',(-20.7113578706468,18.4547273875365,
-1.46640827990993));
#111834=CARTESIAN_POINT('Ctrl Pts',(-20.7164081046749,18.4680662651916,
-1.46724821401887));
#111835=CARTESIAN_POINT('Ctrl Pts',(-20.7217433674324,18.4825998411213,
-1.46815522842632));
#111836=CARTESIAN_POINT('Ctrl Pts',(-20.7221624896271,18.4837446109271,
-1.46822661684574));
#111837=CARTESIAN_POINT('Ctrl Pts',(-20.7225806136401,18.4848897170162,
-1.46829797183507));
#111838=CARTESIAN_POINT('',(-20.8509993841467,19.2126147825168,-0.48905627896718));
#111839=CARTESIAN_POINT('Ctrl Pts',(-20.7225806756345,18.4848898867987,
-1.24458630806144));
#111840=CARTESIAN_POINT('Ctrl Pts',(-20.6661824054662,18.3304332718076,
-1.23372069736793));
#111841=CARTESIAN_POINT('Ctrl Pts',(-20.5919348586647,18.1829508307763,
-1.22298094813775));
#111842=CARTESIAN_POINT('Ctrl Pts',(-20.4894887237695,18.0276123060087,
-1.21154561110675));
#111843=CARTESIAN_POINT('Ctrl Pts',(-20.4774345686897,18.0099242109399,
-1.21024038985349));
#111844=CARTESIAN_POINT('Ctrl Pts',(-20.4603099945566,17.9855970243815,
-1.20844033487475));
#111845=CARTESIAN_POINT('Ctrl Pts',(-20.4554657382646,17.9788010042766,
-1.20793692583058));
#111846=CARTESIAN_POINT('Ctrl Pts',(-20.4470415660747,17.9671293572218,
-1.20707135210583));
#111847=CARTESIAN_POINT('Ctrl Pts',(-20.443480736494,17.9622401368551,-1.20670845761028));
#111848=CARTESIAN_POINT('Ctrl Pts',(-20.4360700664556,17.9521559683733,
-1.2059593064324));
#111849=CARTESIAN_POINT('Ctrl Pts',(-20.432217277546,17.9469632573528,-1.2055731695855));
#111850=CARTESIAN_POINT('Ctrl Pts',(-20.4231497435379,17.9348585065408,
-1.20467212634334));
#111851=CARTESIAN_POINT('Ctrl Pts',(-20.4179162397047,17.9279606130451,
-1.2041579608589));
#111852=CARTESIAN_POINT('Ctrl Pts',(-20.4008334404141,17.9057296134496,
-1.20249840406264));
#111853=CARTESIAN_POINT('Ctrl Pts',(-20.3888156884135,17.8905267612099,
-1.201359675248));
#111854=CARTESIAN_POINT('Ctrl Pts',(-20.3265598744795,17.813956113538,-1.19560103161039));
#111855=CARTESIAN_POINT('Ctrl Pts',(-20.2731079112592,17.7552777134216,
-1.19111372096945));
#111856=CARTESIAN_POINT('Ctrl Pts',(-20.1000689467924,17.5855344376121,
-1.17766518008992));
#111857=CARTESIAN_POINT('Ctrl Pts',(-19.9708586354561,17.4851791348537,
-1.16906415688845));
#111858=CARTESIAN_POINT('Ctrl Pts',(-19.779177507349,17.3689833967405,-1.15653489955564));
#111859=CARTESIAN_POINT('Ctrl Pts',(-19.7255937634343,17.3395937027378,
-1.1530484463857));
#111860=CARTESIAN_POINT('Ctrl Pts',(-19.6626471361593,17.3085314559998,
-1.14888528194358));
#111861=CARTESIAN_POINT('Ctrl Pts',(-19.6544483243733,17.3045512228687,
-1.14834174356928));
#111862=CARTESIAN_POINT('Ctrl Pts',(-19.6421586674782,17.2986827845872,
-1.14752471290199));
#111863=CARTESIAN_POINT('Ctrl Pts',(-19.6380869564036,17.2967544378846,
-1.14725364736495));
#111864=CARTESIAN_POINT('Ctrl Pts',(-19.6307808095641,17.2933227849416,
-1.14676653356237));
#111865=CARTESIAN_POINT('Ctrl Pts',(-19.6275487043282,17.2918146430695,
-1.14655078837474));
#111866=CARTESIAN_POINT('Ctrl Pts',(-19.6205325734518,17.2885623920429,
-1.14608189277962));
#111867=CARTESIAN_POINT('Ctrl Pts',(-19.6167472553636,17.2868213069632,
-1.14582856644096));
#111868=CARTESIAN_POINT('Ctrl Pts',(-19.6061409649053,17.2819807491722,
-1.14511783251206));
#111869=CARTESIAN_POINT('Ctrl Pts',(-19.5993087209995,17.2789063308839,
-1.14465893236172));
#111870=CARTESIAN_POINT('Ctrl Pts',(-19.5591798241623,17.2611044057851,
-1.14195798477386));
#111871=CARTESIAN_POINT('Ctrl Pts',(-19.525526141534,17.2472025131218,-1.1396703469668));
#111872=CARTESIAN_POINT('Ctrl Pts',(-19.4153877701052,17.2049966891448,
-1.13214940977712));
#111873=CARTESIAN_POINT('Ctrl Pts',(-19.3376248017066,17.1802430185681,
-1.12678928356071));
#111874=CARTESIAN_POINT('Ctrl Pts',(-19.0810914400379,17.1146220679987,
-1.10930521312209));
#111875=CARTESIAN_POINT('Ctrl Pts',(-18.89836296349,17.0924428681064,-1.09724057977298));
#111876=CARTESIAN_POINT('Ctrl Pts',(-18.6927243429773,17.0942847882105,
-1.08459114743813));
#111877=CARTESIAN_POINT('Ctrl Pts',(-18.6704139674967,17.0948374722266,
-1.08322948011463));
#111878=CARTESIAN_POINT('Ctrl Pts',(-18.6396296031995,17.096087386524,-1.08136478133196));
#111879=CARTESIAN_POINT('Ctrl Pts',(-18.6311454516231,17.0964830150604,
-1.08085235508817));
#111880=CARTESIAN_POINT('Ctrl Pts',(-18.6165836652113,17.0972499024122,
-1.07997533804089));
#111881=CARTESIAN_POINT('Ctrl Pts',(-18.6105048786102,17.0975963407516,
-1.07960997350805));
#111882=CARTESIAN_POINT('Ctrl Pts',(-18.5979923136674,17.0983636190374,
-1.07885940979585));
#111883=CARTESIAN_POINT('Ctrl Pts',(-18.5915587881476,17.0987876357967,
-1.07847431431837));
#111884=CARTESIAN_POINT('Ctrl Pts',(-18.5766192677292,17.0998408277616,
-1.0775819258605));
#111885=CARTESIAN_POINT('Ctrl Pts',(-18.5681149000994,17.1004920321651,
-1.07707532954861));
#111886=CARTESIAN_POINT('Ctrl Pts',(-18.5410181716267,17.1027317049662,
-1.07546550415896));
#111887=CARTESIAN_POINT('Ctrl Pts',(-18.5224424531343,17.1045146268516,
-1.07436838052141));
#111888=CARTESIAN_POINT('Ctrl Pts',(-18.3441708847962,17.1240073808989,
-1.06389542661839));
#111889=CARTESIAN_POINT('Ctrl Pts',(-18.1869536833619,17.1595972059036,
-1.05514807854796));
#111890=CARTESIAN_POINT('Ctrl Pts',(-17.908489155771,17.2569640080484,-1.0391283317762));
#111891=CARTESIAN_POINT('Ctrl Pts',(-17.7862402686981,17.3132470157437,
-1.03186578695907));
#111892=CARTESIAN_POINT('Ctrl Pts',(-17.6566074513414,17.3885949576223,
-1.0230744383104));
#111893=CARTESIAN_POINT('Ctrl Pts',(-17.6431400224009,17.3966242618457,
-1.02214692552163));
#111894=CARTESIAN_POINT('Ctrl Pts',(-17.6248243605882,17.4078217188635,
-1.02086420744213));
#111895=CARTESIAN_POINT('Ctrl Pts',(-17.6198977230591,17.4108614977312,
-1.02051703991936));
#111896=CARTESIAN_POINT('Ctrl Pts',(-17.6120880690931,17.415724462686,-1.0199632086467));
#111897=CARTESIAN_POINT('Ctrl Pts',(-17.6091968426527,17.4175345020241,
-1.01975740602113));
#111898=CARTESIAN_POINT('Ctrl Pts',(-17.6032369544812,17.4212857434948,
-1.01933155605172));
#111899=CARTESIAN_POINT('Ctrl Pts',(-17.600168920238,17.4232278481787,-1.0191114457333));
#111900=CARTESIAN_POINT('Ctrl Pts',(-17.5928702715098,17.4278743300661,
-1.01858571433786));
#111901=CARTESIAN_POINT('Ctrl Pts',(-17.5886442674297,17.4305858749448,
-1.01827962018844));
#111902=CARTESIAN_POINT('Ctrl Pts',(-17.5744201016722,17.439784174264,-1.01724374439948));
#111903=CARTESIAN_POINT('Ctrl Pts',(-17.5644672952418,17.4463401802521,
-1.01650955102563));
#111904=CARTESIAN_POINT('Ctrl Pts',(-17.540688822463,17.4622927997074,-1.01473383619391));
#111905=CARTESIAN_POINT('Ctrl Pts',(-17.5269182498908,17.4717696959647,
-1.01368766859242));
#111906=CARTESIAN_POINT('Ctrl Pts',(-17.4756936471639,17.5079237954973,
-1.00973299998004));
#111907=CARTESIAN_POINT('Ctrl Pts',(-17.4390016859435,17.5356545857966,
-1.0067721880836));
#111908=CARTESIAN_POINT('Ctrl Pts',(-17.345430048465,17.6112848533801,-0.998936010096704));
#111909=CARTESIAN_POINT('Ctrl Pts',(-17.2901188588802,17.6610252389756,
-0.994012843500479));
#111910=CARTESIAN_POINT('Ctrl Pts',(-17.1277334247407,17.8233055054867,
-0.978845963952766));
#111911=CARTESIAN_POINT('Ctrl Pts',(-17.030311472297,17.9448047966296,-0.968729742295685));
#111912=CARTESIAN_POINT('Ctrl Pts',(-16.9342093851213,18.0960938136812,
-0.957687436261378));
#111913=CARTESIAN_POINT('Ctrl Pts',(-16.9217169768475,18.1165173004625,
-0.95622518042325));
#111914=CARTESIAN_POINT('Ctrl Pts',(-16.9046536568069,18.1455071477022,
-0.954188351445424));
#111915=CARTESIAN_POINT('Ctrl Pts',(-16.8997914923099,18.1538991453648,
-0.953603205203594));
#111916=CARTESIAN_POINT('Ctrl Pts',(-16.8920195688184,18.167528400318,-0.952660008442099));
#111917=CARTESIAN_POINT('Ctrl Pts',(-16.8890741112461,18.172745043666,-0.952300670527777));
#111918=CARTESIAN_POINT('Ctrl Pts',(-16.8829818529425,18.1836427135349,
-0.951553456524428));
#111919=CARTESIAN_POINT('Ctrl Pts',(-16.8798389663413,18.1893258653065,
-0.951165723964566));
#111920=CARTESIAN_POINT('Ctrl Pts',(-16.8724720934962,18.2027930352354,
-0.950251454980925));
#111921=CARTESIAN_POINT('Ctrl Pts',(-16.8682706810135,18.2105893131313,
-0.949725728885034));
#111922=CARTESIAN_POINT('Ctrl Pts',(-16.8544954966124,18.2365396177502,
-0.947987380311746));
#111923=CARTESIAN_POINT('Ctrl Pts',(-16.8451366114532,18.2548068406588,
-0.946782362737516));
#111924=CARTESIAN_POINT('Ctrl Pts',(-16.7969195895766,18.3523910957784,
-0.940438786218297));
#111925=CARTESIAN_POINT('Ctrl Pts',(-16.7627857120895,18.4339500893872,
-0.935466697220141));
#111926=CARTESIAN_POINT('Ctrl Pts',(-16.6909608146935,18.6410770511559,
-0.923366002619506));
#111927=CARTESIAN_POINT('Ctrl Pts',(-16.6596403026142,18.7684487036692,
-0.916388592646102));
#111928=CARTESIAN_POINT('Ctrl Pts',(-16.6347040122347,18.935195888883,-0.907088387874391));
#111929=CARTESIAN_POINT('Ctrl Pts',(-16.6301237574798,18.9726387674235,
-0.904988041061026));
#111930=CARTESIAN_POINT('Ctrl Pts',(-16.6221951274404,19.0558447166839,
-0.900256665875105));
#111931=CARTESIAN_POINT('Ctrl Pts',(-16.6193295473621,19.1016328096204,
-0.89761039489276));
#111932=CARTESIAN_POINT('Ctrl Pts',(-16.6177244726638,19.1550977082651,
-0.894433886191191));
#111933=CARTESIAN_POINT('Ctrl Pts',(-16.6175368056639,19.1627225013456,
-0.893978822287519));
#111934=CARTESIAN_POINT('Ctrl Pts',(-16.6173018807339,19.1749542369422,
-0.893245278152376));
#111935=CARTESIAN_POINT('Ctrl Pts',(-16.6172284502246,19.1795606889306,
-0.892968224132206));
#111936=CARTESIAN_POINT('Ctrl Pts',(-16.6171246645964,19.1877483284721,
-0.89247429639216));
#111937=CARTESIAN_POINT('Ctrl Pts',(-16.6170883596882,19.1913293927005,
-0.892257758631505));
#111938=CARTESIAN_POINT('Ctrl Pts',(-16.6170304167432,19.1989531423377,
-0.891795673294241));
#111939=CARTESIAN_POINT('Ctrl Pts',(-16.6170112720165,19.2029957403879,
-0.891549994801778));
#111940=CARTESIAN_POINT('Ctrl Pts',(-16.6169907240015,19.2139759740558,
-0.890880975854258));
#111941=CARTESIAN_POINT('Ctrl Pts',(-16.6170118446434,19.2209135304453,
-0.890456406001248));
#111942=CARTESIAN_POINT('Ctrl Pts',(-16.6172932451306,19.2562654351253,
-0.888283820471431));
#111943=CARTESIAN_POINT('Ctrl Pts',(-16.6180914884379,19.2846711116209,
-0.88650820891694));
#111944=CARTESIAN_POINT('Ctrl Pts',(-16.6221165596621,19.368072710525,-0.881223467570355));
#111945=CARTESIAN_POINT('Ctrl Pts',(-16.6269184270536,19.422966778176,-0.877654128152968));
#111946=CARTESIAN_POINT('Ctrl Pts',(-16.6514759837071,19.6164141724189,
-0.864883257524241));
#111947=CARTESIAN_POINT('Ctrl Pts',(-16.6828174660238,19.7531458382776,
-0.855531879975794));
#111948=CARTESIAN_POINT('Ctrl Pts',(-16.75623907893,19.9714761807052,-0.840658246436459));
#111949=CARTESIAN_POINT('Ctrl Pts',(-16.7905179086766,20.0552413071479,
-0.83495965037874));
#111950=CARTESIAN_POINT('Ctrl Pts',(-16.8360572771144,20.1489184453406,
-0.828604162730233));
#111951=CARTESIAN_POINT('Ctrl Pts',(-16.8421814937466,20.161210683379,-0.827770418694047));
#111952=CARTESIAN_POINT('Ctrl Pts',(-16.8521957805494,20.1808302295515,
-0.826439833355268));
#111953=CARTESIAN_POINT('Ctrl Pts',(-16.8560099818797,20.1881956249345,
-0.825940349688879));
#111954=CARTESIAN_POINT('Ctrl Pts',(-16.8628597152704,20.2012345346307,
-0.825056113301347));
#111955=CARTESIAN_POINT('Ctrl Pts',(-16.8658779937436,20.2069169492838,
-0.824670757756287));
#111956=CARTESIAN_POINT('Ctrl Pts',(-16.8722212273066,20.2187288451307,
-0.823869686996268));
#111957=CARTESIAN_POINT('Ctrl Pts',(-16.8755506590548,20.2248558441353,
-0.823454136657031));
#111958=CARTESIAN_POINT('Ctrl Pts',(-16.8842769218857,20.2407269561538,
-0.822377583909497));
#111959=CARTESIAN_POINT('Ctrl Pts',(-16.8897205356042,20.2504452050555,
-0.821718259363182));
#111960=CARTESIAN_POINT('Ctrl Pts',(-16.9137060550737,20.292483856465,-0.818865114800046));
#111961=CARTESIAN_POINT('Ctrl Pts',(-16.9330234058495,20.3243557089529,
-0.816699363238438));
#111962=CARTESIAN_POINT('Ctrl Pts',(-16.9865976866517,20.4077018411699,
-0.811013100648686));
#111963=CARTESIAN_POINT('Ctrl Pts',(-17.0222854735611,20.458214648653,-0.807543735795336));
#111964=CARTESIAN_POINT('Ctrl Pts',(-17.1467825047545,20.618998401745,-0.796293123111812));
#111965=CARTESIAN_POINT('Ctrl Pts',(-17.2444281536335,20.7219243089349,
-0.788770462594634));
#111966=CARTESIAN_POINT('Ctrl Pts',(-17.409019288528,20.8638342901307,-0.776740250899853));
#111967=CARTESIAN_POINT('Ctrl Pts',(-17.4690404527405,20.9102085893253,
-0.772457516937216));
#111968=CARTESIAN_POINT('Ctrl Pts',(-17.5392367700206,20.958661364388,-0.767402546046644));
#111969=CARTESIAN_POINT('Ctrl Pts',(-17.5470986426051,20.9640101484255,
-0.766835764205138));
#111970=CARTESIAN_POINT('Ctrl Pts',(-17.5588058980946,20.9718602622615,
-0.765990401295918));
#111971=CARTESIAN_POINT('Ctrl Pts',(-17.5626239318698,20.974402434633,-0.765714494738421));
#111972=CARTESIAN_POINT('Ctrl Pts',(-17.5694371352572,20.9789069987217,
-0.765221710979636));
#111973=CARTESIAN_POINT('Ctrl Pts',(-17.5724290490476,20.9808742180346,
-0.765005161598151));
#111974=CARTESIAN_POINT('Ctrl Pts',(-17.5788815519957,20.9850934072501,
-0.764537805093699));
#111975=CARTESIAN_POINT('Ctrl Pts',(-17.5823436982332,20.987342818405,-0.764286838985219));
#111976=CARTESIAN_POINT('Ctrl Pts',(-17.5919269215151,20.9935293973991,
-0.763591657213845));
#111977=CARTESIAN_POINT('Ctrl Pts',(-17.5980616885217,20.9974451064006,
-0.76314606220414));
#111978=CARTESIAN_POINT('Ctrl Pts',(-17.6319343511103,21.0188203827484,
-0.760683153329686));
#111979=CARTESIAN_POINT('Ctrl Pts',(-17.6600530322491,21.0356645905723,
-0.758629155280327));
#111980=CARTESIAN_POINT('Ctrl Pts',(-17.8308675921068,21.1326732237587,
-0.746147031498064));
#111981=CARTESIAN_POINT('Ctrl Pts',(-17.9820744812969,21.1967201331268,
-0.735129536852101));
#111982=CARTESIAN_POINT('Ctrl Pts',(-18.2489484650775,21.274856427027,-0.716988808393646));
#111983=CARTESIAN_POINT('Ctrl Pts',(-18.3611862289954,21.2980542769874,
-0.709709002545072));
#111984=CARTESIAN_POINT('Ctrl Pts',(-18.4889250262089,21.3138149699519,
-0.701850632073147));
#111985=CARTESIAN_POINT('Ctrl Pts',(-18.5031019853212,21.3154188421148,
-0.700984062011824));
#111986=CARTESIAN_POINT('Ctrl Pts',(-18.525708393466,21.3177451560251,-0.699610903005511));
#111987=CARTESIAN_POINT('Ctrl Pts',(-18.5341276420099,21.318560577904,-0.699101409450835));
#111988=CARTESIAN_POINT('Ctrl Pts',(-18.548995169212,21.3199106367754,-0.698204998522658));
#111989=CARTESIAN_POINT('Ctrl Pts',(-18.5554413934681,21.3204662089711,
-0.6978174289666));
#111990=CARTESIAN_POINT('Ctrl Pts',(-18.5687896234043,21.3215550102637,
-0.697017111803055));
#111991=CARTESIAN_POINT('Ctrl Pts',(-18.5756919082355,21.3220839561022,
-0.696604502964991));
#111992=CARTESIAN_POINT('Ctrl Pts',(-18.5934372164303,21.3233563203803,
-0.695546808775368));
#111993=CARTESIAN_POINT('Ctrl Pts',(-18.604283679647,21.3240501184931,-0.694903282781177));
#111994=CARTESIAN_POINT('Ctrl Pts',(-18.6497615255562,21.3266076329172,
-0.692217031230371));
#111995=CARTESIAN_POINT('Ctrl Pts',(-18.6844318494821,21.3277038002833,
-0.690198340680983));
#111996=CARTESIAN_POINT('Ctrl Pts',(-18.7749971102932,21.3283405967756,
-0.684989197299901));
#111997=CARTESIAN_POINT('Ctrl Pts',(-18.8308754223719,21.326520689323,-0.681839342417253));
#111998=CARTESIAN_POINT('Ctrl Pts',(-19.0845510728595,21.30818490816,-0.66770526995044));
#111999=CARTESIAN_POINT('Ctrl Pts',(-19.2794566785421,21.2661224384763,
-0.657394742607753));
#112000=CARTESIAN_POINT('Ctrl Pts',(-19.4955732415967,21.1865286229346,
-0.644170573043048));
#112001=CARTESIAN_POINT('Ctrl Pts',(-19.5252605407747,21.1748262786256,
-0.642310020563612));
#112002=CARTESIAN_POINT('Ctrl Pts',(-19.560955550427,21.1598150271161,-0.640006098716338));
#112003=CARTESIAN_POINT('Ctrl Pts',(-19.5672279888995,21.157141466583,-0.639598706187977));
#112004=CARTESIAN_POINT('Ctrl Pts',(-19.5775392164593,21.152687428939,-0.638924629426782));
#112005=CARTESIAN_POINT('Ctrl Pts',(-19.5815856015658,21.1509245162147,
-0.638658991695032));
#112006=CARTESIAN_POINT('Ctrl Pts',(-19.5888765445898,21.1477208617822,
-0.638178292201905));
#112007=CARTESIAN_POINT('Ctrl Pts',(-19.5921230212778,21.1462846000402,
-0.637963506611658));
#112008=CARTESIAN_POINT('Ctrl Pts',(-19.5984346187881,21.1434733051312,
-0.637544468857211));
#112009=CARTESIAN_POINT('Ctrl Pts',(-19.6015000361135,21.1420991616646,
-0.63734027919467));
#112010=CARTESIAN_POINT('Ctrl Pts',(-19.6105436869147,21.1380192592625,
-0.636735918907484));
#112011=CARTESIAN_POINT('Ctrl Pts',(-19.6165125589159,21.1352930237778,
-0.636334506879658));
#112012=CARTESIAN_POINT('Ctrl Pts',(-19.6448686053524,21.1221819423287,
-0.634415809423085));
#112013=CARTESIAN_POINT('Ctrl Pts',(-19.6670847067223,21.1114343816403,
-0.632877663218519));
#112014=CARTESIAN_POINT('Ctrl Pts',(-19.7292835658204,21.0799907256176,
-0.628482435917448));
#112015=CARTESIAN_POINT('Ctrl Pts',(-19.768799843259,21.0584047930099,-0.625584594246166));
#112016=CARTESIAN_POINT('Ctrl Pts',(-19.8895240320114,20.987369750416,-0.616462819794181));
#112017=CARTESIAN_POINT('Ctrl Pts',(-19.9681110295935,20.9336998229802,
-0.610137699519105));
#112018=CARTESIAN_POINT('Ctrl Pts',(-20.1606341990481,20.7822639581417,
-0.593981499477576));
#112019=CARTESIAN_POINT('Ctrl Pts',(-20.2682894328901,20.6773313239393,
-0.58430710599027));
#112020=CARTESIAN_POINT('Ctrl Pts',(-20.3729857963497,20.5510053032042,
-0.574291057872095));
#112021=CARTESIAN_POINT('Ctrl Pts',(-20.3818932676913,20.5400359087893,
-0.573432938594564));
#112022=CARTESIAN_POINT('Ctrl Pts',(-20.3959065203289,20.5224213336995,
-0.572073108101216));
#112023=CARTESIAN_POINT('Ctrl Pts',(-20.4010837091802,20.5158337467101,
-0.571568520633174));
#112024=CARTESIAN_POINT('Ctrl Pts',(-20.4101516393898,20.5041534135766,
-0.570680753598069));
#112025=CARTESIAN_POINT('Ctrl Pts',(-20.414058593238,20.4990734427706,-0.570296928178713));
#112026=CARTESIAN_POINT('Ctrl Pts',(-20.4220974030441,20.4885222745632,
-0.569504380690207));
#112027=CARTESIAN_POINT('Ctrl Pts',(-20.4262258736835,20.483048583316,-0.569095795672346));
#112028=CARTESIAN_POINT('Ctrl Pts',(-20.436766166414,20.4689317132398,-0.56804855313326));
#112029=CARTESIAN_POINT('Ctrl Pts',(-20.4431388558035,20.4602594569402,
-0.567411436815932));
#112030=CARTESIAN_POINT('Ctrl Pts',(-20.469546928276,20.4237417762547,-0.564754091978195));
#112031=CARTESIAN_POINT('Ctrl Pts',(-20.4889707980334,20.3954591389648,
-0.562757557265251));
#112032=CARTESIAN_POINT('Ctrl Pts',(-20.5378441393409,20.3204522608832,
-0.557608779161852));
#112033=CARTESIAN_POINT('Ctrl Pts',(-20.5661685036933,20.2730250583122,
-0.554496407991956));
#112034=CARTESIAN_POINT('Ctrl Pts',(-20.6274494475575,20.1606495983284,
-0.547383443430525));
#112035=CARTESIAN_POINT('Ctrl Pts',(-20.6589746514456,20.0950013682202,
-0.543420670502669));
#112036=CARTESIAN_POINT('Ctrl Pts',(-20.7006456271119,19.9953686608852,
-0.537557063547991));
#112037=CARTESIAN_POINT('Ctrl Pts',(-20.7134213668993,19.9625452447437,
-0.535648164490024));
#112038=CARTESIAN_POINT('Ctrl Pts',(-20.7392650272067,19.8909096373497,
-0.531505467693999));
#112039=CARTESIAN_POINT('Ctrl Pts',(-20.752037460671,19.8520067039789,-0.529270205292095));
#112040=CARTESIAN_POINT('Ctrl Pts',(-20.7690474666544,19.7946336295599,
-0.525964916082148));
#112041=CARTESIAN_POINT('Ctrl Pts',(-20.7741781414794,19.7764374674583,
-0.524915331532082));
#112042=CARTESIAN_POINT('Ctrl Pts',(-20.7946963209701,19.6997509089702,
-0.520477600405977));
#112043=CARTESIAN_POINT('Ctrl Pts',(-20.8078159804839,19.6406889783358,
-0.517025262311643));
#112044=CARTESIAN_POINT('Ctrl Pts',(-20.8199723679835,19.5722344460836,
-0.512901190397606));
#112045=CARTESIAN_POINT('Ctrl Pts',(-20.821498830832,19.5633062157223,-0.512360924112629));
#112046=CARTESIAN_POINT('Ctrl Pts',(-20.823694281759,19.5499496480819,-0.51154876385499));
#112047=CARTESIAN_POINT('Ctrl Pts',(-20.8244066116757,19.5455284026217,
-0.511279283813246));
#112048=CARTESIAN_POINT('Ctrl Pts',(-20.8256595644647,19.5375913647195,
-0.510794307785514));
#112049=CARTESIAN_POINT('Ctrl Pts',(-20.8262053588607,19.5340764444796,
-0.510579109141631));
#112050=CARTESIAN_POINT('Ctrl Pts',(-20.827252000903,19.5272221728641,-0.510158628847916));
#112051=CARTESIAN_POINT('Ctrl Pts',(-20.8277537164576,19.5238830074441,
-0.509953403503997));
#112052=CARTESIAN_POINT('Ctrl Pts',(-20.8288494591856,19.5164696311133,
-0.509496951442346));
#112053=CARTESIAN_POINT('Ctrl Pts',(-20.8294395919548,19.5123948705603,
-0.509245509884245));
#112054=CARTESIAN_POINT('Ctrl Pts',(-20.8308794508217,19.5022442397548,
-0.508617812015502));
#112055=CARTESIAN_POINT('Ctrl Pts',(-20.8317146529024,19.496166392462,-0.508240780882291));
#112056=CARTESIAN_POINT('Ctrl Pts',(-20.8356021105131,19.4669354473259,
-0.506422052246403));
#112057=CARTESIAN_POINT('Ctrl Pts',(-20.8382973967367,19.443737509715,-0.504962354972492));
#112058=CARTESIAN_POINT('Ctrl Pts',(-20.8474812586133,19.3513903947303,
-0.499099088402688));
#112059=CARTESIAN_POINT('Ctrl Pts',(-20.8509485244656,19.2819899972872,
-0.494577406431323));
#112060=CARTESIAN_POINT('Ctrl Pts',(-20.8509994310879,19.2125520223715,
-0.490010528127494));
#112061=CARTESIAN_POINT('Ctrl Pts',(-20.8509993841467,19.2126147825168,
-0.48905627896718));
#112062=CARTESIAN_POINT('Ctrl Pts',(-20.8510540322183,19.1409705004862,
-0.484732818607042));
#112063=CARTESIAN_POINT('Ctrl Pts',(-20.8474675455063,19.0691917009212,
-0.480409358246904));
#112064=CARTESIAN_POINT('Ctrl Pts',(-20.8402254628036,18.9976849751246,
-0.476085897886766));
#112065=CARTESIAN_POINT('Ctrl Pts',(-20.8329909785512,18.9262532747475,
-0.471766973735264));
#112066=CARTESIAN_POINT('Ctrl Pts',(-20.8221085499717,18.8550935731786,
-0.467448049583762));
#112067=CARTESIAN_POINT('Ctrl Pts',(-20.80761573801,18.7846119477787,-0.463129125432261));
#112068=CARTESIAN_POINT('Ctrl Pts',(-20.79313335316,18.714181031639,-0.458813308607625));
#112069=CARTESIAN_POINT('Ctrl Pts',(-20.7750458368668,18.6444277090544,
-0.454497491782989));
#112070=CARTESIAN_POINT('Ctrl Pts',(-20.7534422764624,18.5757505277167,
-0.450181674958354));
#112071=CARTESIAN_POINT('Ctrl Pts',(-20.7438446616878,18.5452399489996,
-0.44826432677382));
#112072=CARTESIAN_POINT('Ctrl Pts',(-20.7335537696515,18.514941633152,-0.446346978589286));
#112073=CARTESIAN_POINT('Ctrl Pts',(-20.7225806137986,18.4848897174502,
-0.444429630404752));
#112074=CARTESIAN_POINT('Origin',(18.734,19.211,0.));
#112075=CARTESIAN_POINT('',(16.6170002905278,19.2121090962232,-0.710943720977502));
#112076=CARTESIAN_POINT('Ctrl Pts',(16.7454194503191,18.4848895418526,-0.666446447912836));
#112077=CARTESIAN_POINT('Ctrl Pts',(16.7201110306304,18.55420107782,-0.670880799794245));
#112078=CARTESIAN_POINT('Ctrl Pts',(16.698402847815,18.6249128475929,-0.675315151675655));
#112079=CARTESIAN_POINT('Ctrl Pts',(16.680440926398,18.6966225790074,-0.679749503557064));
#112080=CARTESIAN_POINT('Ctrl Pts',(16.662493389734,18.7682748818904,-0.684180304200555));
#112081=CARTESIAN_POINT('Ctrl Pts',(16.6482862669931,18.8409231094069,-0.688611104844046));
#112082=CARTESIAN_POINT('Ctrl Pts',(16.6379158165232,18.9141497081386,-0.693041905487537));
#112083=CARTESIAN_POINT('Ctrl Pts',(16.6275504637139,18.9873403118716,-0.697470528142895));
#112084=CARTESIAN_POINT('Ctrl Pts',(16.6210181004519,19.0611082624056,-0.701899150798253));
#112085=CARTESIAN_POINT('Ctrl Pts',(16.6183636610493,19.1350271014677,-0.706327773453611));
#112086=CARTESIAN_POINT('Ctrl Pts',(16.6174414214923,19.1607089374613,-0.707866422628241));
#112087=CARTESIAN_POINT('Ctrl Pts',(16.6169868262123,19.1864089348596,-0.709405071802872));
#112088=CARTESIAN_POINT('Ctrl Pts',(16.6170002905278,19.2121090962232,-0.710943720977502));
#112089=CARTESIAN_POINT('Ctrl Pts',(16.6170002428046,19.2120139203676,-0.712619110604606));
#112090=CARTESIAN_POINT('Ctrl Pts',(16.6170721755735,19.3622048615904,-0.721151256465651));
#112091=CARTESIAN_POINT('Ctrl Pts',(16.6331258766371,19.5119663956388,-0.729201744036881));
#112092=CARTESIAN_POINT('Ctrl Pts',(16.6820965468833,19.7382498276167,-0.741816400252578));
#112093=CARTESIAN_POINT('Ctrl Pts',(16.7038575484408,19.8166564320282,-0.746283827984639));
#112094=CARTESIAN_POINT('Ctrl Pts',(16.7417875619102,19.9280069665996,-0.75300998471601));
#112095=CARTESIAN_POINT('Ctrl Pts',(16.7543870689087,19.9620936521435,-0.755123005876484));
#112096=CARTESIAN_POINT('Ctrl Pts',(16.7706293840764,20.0027832821349,-0.757730146936945));
#112097=CARTESIAN_POINT('Ctrl Pts',(16.7734389713608,20.0097148368039,-0.758177289893332));
#112098=CARTESIAN_POINT('Ctrl Pts',(16.7778681013996,20.0204777927027,-0.75887650288154));
#112099=CARTESIAN_POINT('Ctrl Pts',(16.7794623375713,20.0243196340088,-0.759127065838273));
#112100=CARTESIAN_POINT('Ctrl Pts',(16.7824436436943,20.0314446914402,-0.759593622265121));
#112101=CARTESIAN_POINT('Ctrl Pts',(16.7838276867843,20.0347291130496,-0.75980943151961));
#112102=CARTESIAN_POINT('Ctrl Pts',(16.7869797398919,20.0421566627409,-0.760299146739663));
#112103=CARTESIAN_POINT('Ctrl Pts',(16.7887526763491,20.0462976357273,-0.760573349045485));
#112104=CARTESIAN_POINT('Ctrl Pts',(16.794151598636,20.0587972605664,-0.761404532062207));
#112105=CARTESIAN_POINT('Ctrl Pts',(16.7978182879772,20.0671380650843,-0.761963907066338));
#112106=CARTESIAN_POINT('Ctrl Pts',(16.8264545300996,20.13115348135,-0.766292207608628));
#112107=CARTESIAN_POINT('Ctrl Pts',(16.853764529941,20.1857436858668,-0.770187814146948));
#112108=CARTESIAN_POINT('Ctrl Pts',(16.9113896732437,20.2894733572407,-0.777892465160095));
#112109=CARTESIAN_POINT('Ctrl Pts',(16.9414352247186,20.3387075234899,-0.781691412437072));
#112110=CARTESIAN_POINT('Ctrl Pts',(17.034267564791,20.4777246916938,-0.792733422523316));
#112111=CARTESIAN_POINT('Ctrl Pts',(17.1020634321017,20.5639480019873,-0.799975476567422));
#112112=CARTESIAN_POINT('Ctrl Pts',(17.2136539678244,20.6852086621884,-0.81056922548381));
#112113=CARTESIAN_POINT('Ctrl Pts',(17.2526575030984,20.7243963366687,-0.814069183085821));
#112114=CARTESIAN_POINT('Ctrl Pts',(17.309882590848,20.7775567411757,-0.818924447556188));
#112115=CARTESIAN_POINT('Ctrl Pts',(17.3268631398915,20.7928268991362,-0.820332738954798));
#112116=CARTESIAN_POINT('Ctrl Pts',(17.3532541641535,20.8157983089728,-0.822472985443773));
#112117=CARTESIAN_POINT('Ctrl Pts',(17.3624890431794,20.8236978578387,-0.823213077882509));
#112118=CARTESIAN_POINT('Ctrl Pts',(17.3797349967899,20.838194820665,-0.824579076934076));
#112119=CARTESIAN_POINT('Ctrl Pts',(17.3877275052182,20.8448136549541,-0.825205849827082));
#112120=CARTESIAN_POINT('Ctrl Pts',(17.4009524691374,20.8556026997506,-0.826232775485803));
#112121=CARTESIAN_POINT('Ctrl Pts',(17.4061565314278,20.8598072913878,-0.826634317755328));
#112122=CARTESIAN_POINT('Ctrl Pts',(17.4164195138048,20.8680191038776,-0.827421239841784));
#112123=CARTESIAN_POINT('Ctrl Pts',(17.4214769952318,20.872027998438,-0.827806684392119));
#112124=CARTESIAN_POINT('Ctrl Pts',(17.4331770167175,20.8812154065039,-0.828693042407577));
#112125=CARTESIAN_POINT('Ctrl Pts',(17.4398323152578,20.8863775529277,-0.8291933012266));
#112126=CARTESIAN_POINT('Ctrl Pts',(17.4577691339486,20.9001194909548,-0.830531204646337));
#112127=CARTESIAN_POINT('Ctrl Pts',(17.4691064243091,20.9086260291679,-0.831365970496308));
#112128=CARTESIAN_POINT('Ctrl Pts',(17.5673788772651,20.980830251459,-0.838511190985972));
#112129=CARTESIAN_POINT('Ctrl Pts',(17.658980633666,21.0379213769114,-0.844555606789997));
#112130=CARTESIAN_POINT('Ctrl Pts',(17.9003338187212,21.1638782901066,-0.859509511383662));
#112131=CARTESIAN_POINT('Ctrl Pts',(18.0544765438377,21.2227082675158,-0.868183303358356));
#112132=CARTESIAN_POINT('Ctrl Pts',(18.2518193841745,21.2727285920438,-0.879791342789503));
#112133=CARTESIAN_POINT('Ctrl Pts',(18.2900413229699,21.28129543473,-0.882064101689193));
#112134=CARTESIAN_POINT('Ctrl Pts',(18.3359843080636,21.2902621362035,-0.884848709101056));
#112135=CARTESIAN_POINT('Ctrl Pts',(18.3435003741053,21.2916868001242,-0.885305933870731));
#112136=CARTESIAN_POINT('Ctrl Pts',(18.3551553850479,21.2938306231413,-0.886017766370994));
#112137=CARTESIAN_POINT('Ctrl Pts',(18.3592891154542,21.2945782680939,-0.886270783978306));
#112138=CARTESIAN_POINT('Ctrl Pts',(18.3669338506184,21.2959374434686,-0.886739763218027));
#112139=CARTESIAN_POINT('Ctrl Pts',(18.3704441847306,21.29655241359,-0.88695552682346));
#112140=CARTESIAN_POINT('Ctrl Pts',(18.3783518622324,21.2979171762964,-0.887442508573786));
#112141=CARTESIAN_POINT('Ctrl Pts',(18.3827500025938,21.2986619307488,-0.887714006478885));
#112142=CARTESIAN_POINT('Ctrl Pts',(18.3940282459288,21.3005350716878,-0.888411809653817));
#112143=CARTESIAN_POINT('Ctrl Pts',(18.4009115669748,21.3016433703701,-0.888839211734882));
#112144=CARTESIAN_POINT('Ctrl Pts',(18.4415321412924,21.3079780811404,-0.891369892077375));
#112145=CARTESIAN_POINT('Ctrl Pts',(18.4753843176729,21.3124214579499,-0.893513182270694));
#112146=CARTESIAN_POINT('Ctrl Pts',(18.5262581163844,21.3178512632335,-0.896770859022912));
#112147=CARTESIAN_POINT('Ctrl Pts',(18.5432102147203,21.3194539748645,-0.897862463120768));
#112148=CARTESIAN_POINT('Ctrl Pts',(18.5665359734006,21.3213756728581,-0.899371291000689));
#112149=CARTESIAN_POINT('Ctrl Pts',(18.5728948702985,21.3218706300148,-0.899783310766908));
#112150=CARTESIAN_POINT('Ctrl Pts',(18.731701388198,21.3335098807761,-0.910088948362018));
#112151=CARTESIAN_POINT('Ctrl Pts',(18.8849097070059,21.328140398447,-0.920354509541062));
#112152=CARTESIAN_POINT('Ctrl Pts',(19.1280848751859,21.2930668979692,-0.936300611875996));
#112153=CARTESIAN_POINT('Ctrl Pts',(19.2189970957486,21.2737862735516,-0.942191090915608));
#112154=CARTESIAN_POINT('Ctrl Pts',(19.3286539598942,21.2428760308616,-0.949187136634125));
#112155=CARTESIAN_POINT('Ctrl Pts',(19.3488611490825,21.2368527475187,-0.95047202656592));
#112156=CARTESIAN_POINT('Ctrl Pts',(19.3775209093902,21.2278416102537,-0.95228877618808));
#112157=CARTESIAN_POINT('Ctrl Pts',(19.3860492057119,21.2251005632437,-0.952828676750796));
#112158=CARTESIAN_POINT('Ctrl Pts',(19.4007516765177,21.2202719264654,-0.953758290330705));
#112159=CARTESIAN_POINT('Ctrl Pts',(19.406934031911,21.2182098203206,-0.954148836193282));
#112160=CARTESIAN_POINT('Ctrl Pts',(19.4187669317587,21.2142021767488,-0.95489568860466));
#112161=CARTESIAN_POINT('Ctrl Pts',(19.424418944651,21.2122612007821,-0.955252141450639));
#112162=CARTESIAN_POINT('Ctrl Pts',(19.4391247784187,21.2071413081171,-0.956178890925988));
#112163=CARTESIAN_POINT('Ctrl Pts',(19.4481654042787,21.2039246987908,-0.956747933098307));
#112164=CARTESIAN_POINT('Ctrl Pts',(19.4790725825043,21.1926907567521,-0.958691199611591));
#112165=CARTESIAN_POINT('Ctrl Pts',(19.5008290278612,21.1843739417313,-0.96005544967437));
#112166=CARTESIAN_POINT('Ctrl Pts',(19.6812591892358,21.111966351105,-0.971349389867178));
#112167=CARTESIAN_POINT('Ctrl Pts',(19.8317602969987,21.0292140245565,-0.980570870939259));
#112168=CARTESIAN_POINT('Ctrl Pts',(20.0438205499428,20.8765876721058,-0.99477769771984));
#112169=CARTESIAN_POINT('Ctrl Pts',(20.1135298459832,20.8193242800664,-0.999702041086007));
#112170=CARTESIAN_POINT('Ctrl Pts',(20.2075785076758,20.7314425783718,-1.00704526893611));
#112171=CARTESIAN_POINT('Ctrl Pts',(20.2350564296684,20.7043212731197,-1.00928633988184));
#112172=CARTESIAN_POINT('Ctrl Pts',(20.2670472697989,20.6709702266446,-1.0120356762018));
#112173=CARTESIAN_POINT('Ctrl Pts',(20.2722891401027,20.6654461184853,-1.0124908582202));
#112174=CARTESIAN_POINT('Ctrl Pts',(20.2803697489133,20.656837877807,-1.01320008194604));
#112175=CARTESIAN_POINT('Ctrl Pts',(20.283229385846,20.6537733289009,-1.01345254967954));
#112176=CARTESIAN_POINT('Ctrl Pts',(20.2885027108963,20.6480883808154,-1.01392090825715));
#112177=CARTESIAN_POINT('Ctrl Pts',(20.2909188927957,20.6454703737422,-1.01413660375317));
#112178=CARTESIAN_POINT('Ctrl Pts',(20.2963498763317,20.6395558511298,-1.01462391342197));
#112179=CARTESIAN_POINT('Ctrl Pts',(20.2993608403056,20.6362559049736,-1.01489581029872));
#112180=CARTESIAN_POINT('Ctrl Pts',(20.3081696001938,20.6265401257491,-1.01569629101565));
#112181=CARTESIAN_POINT('Ctrl Pts',(20.3139384751181,20.6200983595085,-1.01622696985406));
#112182=CARTESIAN_POINT('Ctrl Pts',(20.3539129043045,20.5749071551173,-1.01994833415176));
#112183=CARTESIAN_POINT('Ctrl Pts',(20.3867259501602,20.5349548807027,-1.0232301831665));
#112184=CARTESIAN_POINT('Ctrl Pts',(20.4313964331169,20.4763142183867,-1.02798925885708));
#112185=CARTESIAN_POINT('Ctrl Pts',(20.4444766487415,20.4585753722496,-1.02942175511493));
#112186=CARTESIAN_POINT('Ctrl Pts',(20.4839563367759,20.4032464403743,-1.03386105231835));
#112187=CARTESIAN_POINT('Ctrl Pts',(20.5094109551861,20.3649993504169,-1.03688946022074));
#112188=CARTESIAN_POINT('Ctrl Pts',(20.5911954386698,20.2329946161385,-1.04714744045571));
#112189=CARTESIAN_POINT('Ctrl Pts',(20.6415049234467,20.1357033724387,-1.05437842966978));
#112190=CARTESIAN_POINT('Ctrl Pts',(20.7055081559617,19.9842253924476,-1.06494830594674));
#112191=CARTESIAN_POINT('Ctrl Pts',(20.7249562597562,19.9326757639309,-1.06843560131803));
#112192=CARTESIAN_POINT('Ctrl Pts',(20.7532158563074,19.847892532634,-1.07399051610733));
#112193=CARTESIAN_POINT('Ctrl Pts',(20.7632671672991,19.8151024352732,-1.07609653604523));
#112194=CARTESIAN_POINT('Ctrl Pts',(20.7754329805161,19.7716756249597,-1.07883208803829));
#112195=CARTESIAN_POINT('Ctrl Pts',(20.7782683399662,19.7612478817376,-1.07948494525895));
#112196=CARTESIAN_POINT('Ctrl Pts',(20.7827823683459,19.7441297914933,-1.08055023107254));
#112197=CARTESIAN_POINT('Ctrl Pts',(20.7845083788725,19.7374522365306,-1.08096418850021));
#112198=CARTESIAN_POINT('Ctrl Pts',(20.7877868232135,19.7245079014751,-1.08176359176459));
#112199=CARTESIAN_POINT('Ctrl Pts',(20.7893432811271,19.7182422283619,-1.08214916383628));
#112200=CARTESIAN_POINT('Ctrl Pts',(20.7928716554397,19.7037554954688,-1.08303750604323));
#112201=CARTESIAN_POINT('Ctrl Pts',(20.7948230459075,19.6955295125245,-1.08353961001947));
#112202=CARTESIAN_POINT('Ctrl Pts',(20.7999401110022,19.6733685283922,-1.08488618416961));
#112203=CARTESIAN_POINT('Ctrl Pts',(20.8030140914805,19.6594126475277,-1.08572771234218));
#112204=CARTESIAN_POINT('Ctrl Pts',(20.8299391557904,19.5309966753832,-1.09341428843042));
#112205=CARTESIAN_POINT('Ctrl Pts',(20.844412813131,19.4147691027026,-1.09994213320598));
#112206=CARTESIAN_POINT('Ctrl Pts',(20.8559026263753,19.1351854659258,-1.11526004969816));
#112207=CARTESIAN_POINT('Ctrl Pts',(20.8437863383083,18.9722359259568,-1.12386685462392));
#112208=CARTESIAN_POINT('Ctrl Pts',(20.8070320844516,18.7805683776233,-1.13507490368345));
#112209=CARTESIAN_POINT('Ctrl Pts',(20.8002202035693,18.7489748729143,-1.1369600696242));
#112210=CARTESIAN_POINT('Ctrl Pts',(20.7910040818629,18.7105248052916,-1.13931433290164));
#112211=CARTESIAN_POINT('Ctrl Pts',(20.7892838746561,18.7035067444061,-1.13974650713986));
#112212=CARTESIAN_POINT('Ctrl Pts',(20.7865298195019,18.6925145111395,-1.14042747868541));
#112213=CARTESIAN_POINT('Ctrl Pts',(20.7855202608741,18.6885342301473,-1.14067489660744));
#112214=CARTESIAN_POINT('Ctrl Pts',(20.783610814994,18.6810969258929,-1.14113881843456));
#112215=CARTESIAN_POINT('Ctrl Pts',(20.7827137559631,18.6776392343322,-1.14135515815387));
#112216=CARTESIAN_POINT('Ctrl Pts',(20.7806451001205,18.6697478737409,-1.14185039413272));
#112217=CARTESIAN_POINT('Ctrl Pts',(20.7794678494619,18.6653157452054,-1.142129613848));
#112218=CARTESIAN_POINT('Ctrl Pts',(20.7758018722212,18.6516925855068,-1.14299109027105));
#112219=CARTESIAN_POINT('Ctrl Pts',(20.7732655681816,18.6425146405063,-1.14357600012887));
#112220=CARTESIAN_POINT('Ctrl Pts',(20.7494659901649,18.5586019094306,-1.14896334844942));
#112221=CARTESIAN_POINT('Ctrl Pts',(20.7241672868575,18.4850813388748,-1.15397009932529));
#112222=CARTESIAN_POINT('Ctrl Pts',(20.6794752132422,18.3752441480921,-1.16173125821361));
#112223=CARTESIAN_POINT('Ctrl Pts',(20.6629669607468,18.3378173233877,-1.16442839640459));
#112224=CARTESIAN_POINT('Ctrl Pts',(20.5983938453691,18.2022023902509,-1.17435057158121));
#112225=CARTESIAN_POINT('Ctrl Pts',(20.5438256344561,18.1072918553061,-1.18157787902276));
#112226=CARTESIAN_POINT('Ctrl Pts',(20.4511414351924,17.9715886342431,-1.19214007518589));
#112227=CARTESIAN_POINT('Ctrl Pts',(20.418354422777,17.9273854792938,-1.19562337147695));
#112228=CARTESIAN_POINT('Ctrl Pts',(20.3624109825724,17.8578035399774,-1.20117276493636));
#112229=CARTESIAN_POINT('Ctrl Pts',(20.3402957503356,17.8316243566024,-1.20327715677248));
#112230=CARTESIAN_POINT('Ctrl Pts',(20.3103831304053,17.7979104915539,-1.20601101777612));
#112231=CARTESIAN_POINT('Ctrl Pts',(20.3031506873816,17.7898835868325,-1.2066637692684));
#112232=CARTESIAN_POINT('Ctrl Pts',(20.2912009041653,17.7768236098939,-1.20772897911582));
#112233=CARTESIAN_POINT('Ctrl Pts',(20.2865199210203,17.7717576748657,-1.20814296503141));
#112234=CARTESIAN_POINT('Ctrl Pts',(20.2774086597171,17.7619933025391,-1.20894249053427));
#112235=CARTESIAN_POINT('Ctrl Pts',(20.2729814833772,17.7572920873077,-1.20932815602549));
#112236=CARTESIAN_POINT('Ctrl Pts',(20.2627063204704,17.74648044752,-1.2102168102565));
#112237=CARTESIAN_POINT('Ctrl Pts',(20.256843063044,17.7403846382049,-1.21071913203689));
#112238=CARTESIAN_POINT('Ctrl Pts',(20.2409688782791,17.7240775808132,-1.2120665077803));
#112239=CARTESIAN_POINT('Ctrl Pts',(20.2308906531443,17.7139322432663,-1.21290861546797));
#112240=CARTESIAN_POINT('Ctrl Pts',(20.1369968128611,17.6213093453177,-1.22063510567093));
#112241=CARTESIAN_POINT('Ctrl Pts',(20.0465437660938,17.5458421600769,-1.22719840370218));
#112242=CARTESIAN_POINT('Ctrl Pts',(19.8163415546447,17.3842530644563,-1.24259187359711));
#112243=CARTESIAN_POINT('Ctrl Pts',(19.6719714362308,17.3060945328849,-1.25123869641716));
#112244=CARTESIAN_POINT('Ctrl Pts',(19.4912802674861,17.2338362297299,-1.26243140406671));
#112245=CARTESIAN_POINT('Ctrl Pts',(19.4622491643232,17.222960034575,-1.26424160000635));
#112246=CARTESIAN_POINT('Ctrl Pts',(19.4262575064435,17.2103702390641,-1.26651244218093));
#112247=CARTESIAN_POINT('Ctrl Pts',(19.4195117344216,17.2080487888513,-1.26693919539804));
#112248=CARTESIAN_POINT('Ctrl Pts',(19.4088835199112,17.2044512376676,-1.26761353814391));
#112249=CARTESIAN_POINT('Ctrl Pts',(19.4050088242724,17.2031521825187,-1.26785979304073));
#112250=CARTESIAN_POINT('Ctrl Pts',(19.397736900938,17.2007375514422,-1.26832277146825));
#112251=CARTESIAN_POINT('Ctrl Pts',(19.3943406001685,17.1996193605286,-1.26853933829952));
#112252=CARTESIAN_POINT('Ctrl Pts',(19.3865516676927,17.1970768026022,-1.26903676250137));
#112253=CARTESIAN_POINT('Ctrl Pts',(19.3821572105583,17.1956582043003,-1.26931795407472));
#112254=CARTESIAN_POINT('Ctrl Pts',(19.3685310777802,17.1913086557225,-1.27019147997714));
#112255=CARTESIAN_POINT('Ctrl Pts',(19.3592840547534,17.1884267238223,-1.270786573982));
#112256=CARTESIAN_POINT('Ctrl Pts',(19.2481012735029,17.1546107590281,-1.27796653456379));
#112257=CARTESIAN_POINT('Ctrl Pts',(19.144001982154,17.1313534392421,-1.28493125873903));
#112258=CARTESIAN_POINT('Ctrl Pts',(18.9302864243071,17.1002791382127,-1.29917768219238));
#112259=CARTESIAN_POINT('Ctrl Pts',(18.8208977152644,17.0929531387274,-1.30643903080193));
#112260=CARTESIAN_POINT('Ctrl Pts',(18.6488171391698,17.0947879134385,-1.31756399007033));
#112261=CARTESIAN_POINT('Ctrl Pts',(18.5862613574716,17.0982330510975,-1.32154890782154));
#112262=CARTESIAN_POINT('Ctrl Pts',(18.4991728130932,17.106917069951,-1.32700390776245));
#112263=CARTESIAN_POINT('Ctrl Pts',(18.474444925285,17.1098241317021,-1.32854246718625));
#112264=CARTESIAN_POINT('Ctrl Pts',(18.4312397297831,17.1156778256324,-1.33121311773824));
#112265=CARTESIAN_POINT('Ctrl Pts',(18.4127398793921,17.1184344058632,-1.33235098995107));
#112266=CARTESIAN_POINT('Ctrl Pts',(18.3858541005302,17.1228054977378,-1.33399682884304));
#112267=CARTESIAN_POINT('Ctrl Pts',(18.3774379562992,17.1242260882117,-1.33451091157527));
#112268=CARTESIAN_POINT('Ctrl Pts',(18.3626808183819,17.1268088812865,-1.33541041996459));
#112269=CARTESIAN_POINT('Ctrl Pts',(18.3563361561911,17.1279492141412,-1.33579653505552));
#112270=CARTESIAN_POINT('Ctrl Pts',(18.3440143594684,17.1302219708145,-1.33654523218482));
#112271=CARTESIAN_POINT('Ctrl Pts',(18.3380367089998,17.1313512123604,-1.33690791134002));
#112272=CARTESIAN_POINT('Ctrl Pts',(18.3237390948993,17.1341160637259,-1.33777414333123));
#112273=CARTESIAN_POINT('Ctrl Pts',(18.3154238858244,17.1357759314167,-1.33827691900606));
#112274=CARTESIAN_POINT('Ctrl Pts',(18.2853390465207,17.1419695964793,-1.34009251807192));
#112275=CARTESIAN_POINT('Ctrl Pts',(18.2636307342855,17.1467964560217,-1.34139598784263));
#112276=CARTESIAN_POINT('Ctrl Pts',(18.0627498736254,17.1947961193728,-1.35340656131926));
#112277=CARTESIAN_POINT('Ctrl Pts',(17.8898625021901,17.2608479974272,-1.36327108162538));
#112278=CARTESIAN_POINT('Ctrl Pts',(17.6564401292847,17.3869620717287,-1.37773038284321));
#112279=CARTESIAN_POINT('Ctrl Pts',(17.587451897218,17.4295188653848,-1.38218214560317));
#112280=CARTESIAN_POINT('Ctrl Pts',(17.4913585237652,17.4966937421309,-1.38888705149075));
#112281=CARTESIAN_POINT('Ctrl Pts',(17.4621807076068,17.5182273877247,-1.39099578831577));
#112282=CARTESIAN_POINT('Ctrl Pts',(17.4276698142784,17.5450929207151,-1.39359843021575));
#112283=CARTESIAN_POINT('Ctrl Pts',(17.4217918922038,17.5497189193321,-1.39404561885559));
#112284=CARTESIAN_POINT('Ctrl Pts',(17.4126815777818,17.5569673667819,-1.39474504477035));
#112285=CARTESIAN_POINT('Ctrl Pts',(17.4094321284608,17.5595684156936,-1.39499577711186));
#112286=CARTESIAN_POINT('Ctrl Pts',(17.4034133886956,17.5644153581116,-1.39546258589766));
#112287=CARTESIAN_POINT('Ctrl Pts',(17.4006420937703,17.5666586709635,-1.39567847765864));
#112288=CARTESIAN_POINT('Ctrl Pts',(17.394381039644,17.5717531155132,-1.39616838630699));
#112289=CARTESIAN_POINT('Ctrl Pts',(17.3908947269368,17.57460838066,-1.39644269930387));
#112290=CARTESIAN_POINT('Ctrl Pts',(17.3806056010608,17.5830901324146,-1.39725671602911));
#112291=CARTESIAN_POINT('Ctrl Pts',(17.3738289347408,17.5887479841084,-1.39779861968202));
#112292=CARTESIAN_POINT('Ctrl Pts',(17.3242111151522,17.6307034491885,-1.40180779530323));
#112293=CARTESIAN_POINT('Ctrl Pts',(17.2827975181789,17.6686472326923,-1.4053825531971));
#112294=CARTESIAN_POINT('Ctrl Pts',(17.1985945891666,17.7521914187054,-1.4130622312626));
#112295=CARTESIAN_POINT('Ctrl Pts',(17.156215584395,17.7981348345008,-1.41717754863527));
#112296=CARTESIAN_POINT('Ctrl Pts',(17.045248180235,17.9296640609522,-1.42854451615834));
#112297=CARTESIAN_POINT('Ctrl Pts',(16.9811727702815,18.018815173926,-1.43579412729792));
#112298=CARTESIAN_POINT('Ctrl Pts',(16.8955511350191,18.1598758862508,-1.44640312640984));
#112299=CARTESIAN_POINT('Ctrl Pts',(16.8686818008557,18.2083310713638,-1.44991077271153));
#112300=CARTESIAN_POINT('Ctrl Pts',(16.8282391802368,18.2885304115173,-1.45549435156725));
#112301=CARTESIAN_POINT('Ctrl Pts',(16.8134880391355,18.3196479535453,-1.45760917390799));
#112302=CARTESIAN_POINT('Ctrl Pts',(16.7951057262466,18.3610028643832,-1.46035435937222));
#112303=CARTESIAN_POINT('Ctrl Pts',(16.7907855005412,18.3709264608044,-1.46100824951286));
#112304=CARTESIAN_POINT('Ctrl Pts',(16.7838354404969,18.3872313332866,-1.46207481943634));
#112305=CARTESIAN_POINT('Ctrl Pts',(16.7811604121196,18.393593019872,-1.46248903467034));
#112306=CARTESIAN_POINT('Ctrl Pts',(16.7760434443961,18.4059305633697,-1.46328865919097));
#112307=CARTESIAN_POINT('Ctrl Pts',(16.773597639742,18.4119047248618,-1.46367419617511));
#112308=CARTESIAN_POINT('Ctrl Pts',(16.7680147562702,18.4257214720483,-1.46456206307928));
#112309=CARTESIAN_POINT('Ctrl Pts',(16.7648971981634,18.4335718657141,-1.46506372953812));
#112310=CARTESIAN_POINT('Ctrl Pts',(16.7566421298026,18.4547273863516,-1.46640825726746));
#112311=CARTESIAN_POINT('Ctrl Pts',(16.7515918955811,18.4680662644982,-1.46724819140767));
#112312=CARTESIAN_POINT('Ctrl Pts',(16.7462566540906,18.4825997824912,-1.46815520219957));
#112313=CARTESIAN_POINT('Ctrl Pts',(16.7458375532442,18.4837444938304,-1.46822658697579));
#112314=CARTESIAN_POINT('Ctrl Pts',(16.7454194504776,18.4848895414187,-1.46829793832533));
#112315=CARTESIAN_POINT('',(16.617000615792,19.2126147021618,-0.489056278967189));
#112316=CARTESIAN_POINT('Ctrl Pts',(16.7454193884829,18.4848897112021,-1.2445862186816));
#112317=CARTESIAN_POINT('Ctrl Pts',(16.8018177025919,18.3304330182041,-1.23372060137579));
#112318=CARTESIAN_POINT('Ctrl Pts',(16.8760653119355,18.1829505081514,-1.22298084578471));
#112319=CARTESIAN_POINT('Ctrl Pts',(16.9785115262827,18.027611935167,-1.21154550356326));
#112320=CARTESIAN_POINT('Ctrl Pts',(16.9905656820716,18.0099238470398,-1.21024028263197));
#112321=CARTESIAN_POINT('Ctrl Pts',(17.0076902571063,17.9855966698589,-1.20844022807956));
#112322=CARTESIAN_POINT('Ctrl Pts',(17.0125345137391,17.9788006522226,-1.20793681914285));
#112323=CARTESIAN_POINT('Ctrl Pts',(17.020958686521,17.9671290093565,-1.20707124559801));
#112324=CARTESIAN_POINT('Ctrl Pts',(17.0245195163649,17.9622397907119,-1.20670835117514));
#112325=CARTESIAN_POINT('Ctrl Pts',(17.0319301869605,17.9521556257385,-1.20595920014336));
#112326=CARTESIAN_POINT('Ctrl Pts',(17.0357829761629,17.9469629165046,-1.20557306336987));
#112327=CARTESIAN_POINT('Ctrl Pts',(17.0448505108803,17.934858169794,-1.20467202029334));
#112328=CARTESIAN_POINT('Ctrl Pts',(17.0500840151204,17.9279602786125,-1.20415785490094));
#112329=CARTESIAN_POINT('Ctrl Pts',(17.0671668158501,17.905729286248,-1.20249829838223));
#112330=CARTESIAN_POINT('Ctrl Pts',(17.0791845688017,17.8905264389161,-1.20135956975118));
#112331=CARTESIAN_POINT('Ctrl Pts',(17.1414403898606,17.8139558127088,-1.19560092677479));
#112332=CARTESIAN_POINT('Ctrl Pts',(17.1948923580414,17.7552774291804,-1.19111361657809));
#112333=CARTESIAN_POINT('Ctrl Pts',(17.3679313906468,17.5855341478621,-1.17766507248548));
#112334=CARTESIAN_POINT('Ctrl Pts',(17.4971417734192,17.4851788360257,-1.1690640459197));
#112335=CARTESIAN_POINT('Ctrl Pts',(17.6888228829003,17.368983179271,-1.15653479048417));
#112336=CARTESIAN_POINT('Ctrl Pts',(17.7424065273263,17.339593552571,-1.15304834380677));
#112337=CARTESIAN_POINT('Ctrl Pts',(17.8053530477427,17.3085313662473,-1.14888518660732));
#112338=CARTESIAN_POINT('Ctrl Pts',(17.8135518570711,17.304551135281,-1.14834164841957));
#112339=CARTESIAN_POINT('Ctrl Pts',(17.8258415114177,17.2986826996303,-1.14752461795865));
#112340=CARTESIAN_POINT('Ctrl Pts',(17.8299132224218,17.296754353427,-1.14725355243867));
#112341=CARTESIAN_POINT('Ctrl Pts',(17.8372193709518,17.2933227005219,-1.14676643854585));
#112342=CARTESIAN_POINT('Ctrl Pts',(17.8404514779532,17.2918145581983,-1.14655069325011));
#112343=CARTESIAN_POINT('Ctrl Pts',(17.8474676156369,17.288562304833,-1.14608179722227));
#112344=CARTESIAN_POINT('Ctrl Pts',(17.8512529387803,17.2868212178851,-1.14582847055763));
#112345=CARTESIAN_POINT('Ctrl Pts',(17.8618592457823,17.2819806538693,-1.14511773555571));
#112346=CARTESIAN_POINT('Ctrl Pts',(17.8686915012149,17.2789062313153,-1.14465883465491));
#112347=CARTESIAN_POINT('Ctrl Pts',(17.9088205167704,17.261104259353,-1.1419578792227));
#112348=CARTESIAN_POINT('Ctrl Pts',(17.9424743087865,17.2472023294799,-1.13967023409614));
#112349=CARTESIAN_POINT('Ctrl Pts',(18.0526131915964,17.2049963454243,-1.1321492625559));
#112350=CARTESIAN_POINT('Ctrl Pts',(18.1303765751753,17.1802425924568,-1.12678910835977));
#112351=CARTESIAN_POINT('Ctrl Pts',(18.3869095020089,17.11462199314,-1.10930507321492));
#112352=CARTESIAN_POINT('Ctrl Pts',(18.5696370501885,17.0924429474123,-1.0972405059824));
#112353=CARTESIAN_POINT('Ctrl Pts',(18.7752748015699,17.0942847709101,-1.08459112651074));
#112354=CARTESIAN_POINT('Ctrl Pts',(18.7975852360155,17.0948374476744,-1.0832294555494));
#112355=CARTESIAN_POINT('Ctrl Pts',(18.8283696716387,17.0960873541174,-1.08136475242817));
#112356=CARTESIAN_POINT('Ctrl Pts',(18.8368538355264,17.096482980337,-1.08085232543775));
#112357=CARTESIAN_POINT('Ctrl Pts',(18.8514156400355,17.0972498638032,-1.07997530729859));
#112358=CARTESIAN_POINT('Ctrl Pts',(18.8574944324195,17.0975963004759,-1.07960994241799));
#112359=CARTESIAN_POINT('Ctrl Pts',(18.87000700651,17.0983635752619,-1.07885937815799));
#112360=CARTESIAN_POINT('Ctrl Pts',(18.8764405353957,17.0987875901687,-1.07847428247985));
#112361=CARTESIAN_POINT('Ctrl Pts',(18.8913800590137,17.0998407775738,-1.07758189383363));
#112362=CARTESIAN_POINT('Ctrl Pts',(18.899884426487,17.1004919792367,-1.07707529753252));
#112363=CARTESIAN_POINT('Ctrl Pts',(18.9269811360591,17.1027316417658,-1.07546547327035));
#112364=CARTESIAN_POINT('Ctrl Pts',(18.9455568359123,17.1045145556207,-1.07436835073024));
#112365=CARTESIAN_POINT('Ctrl Pts',(19.1238252816247,17.1240069056998,-1.06389558019926));
#112366=CARTESIAN_POINT('Ctrl Pts',(19.2810394936595,17.159595631502,-1.05514838677631));
#112367=CARTESIAN_POINT('Ctrl Pts',(19.559504417885,17.2569610830505,-1.03912864398778));
#112368=CARTESIAN_POINT('Ctrl Pts',(19.6817562466483,17.3132450592697,-1.03186594805774));
#112369=CARTESIAN_POINT('Ctrl Pts',(19.8113918692138,17.388594554649,-1.02307441343735));
#112370=CARTESIAN_POINT('Ctrl Pts',(19.8248594297125,17.396623931143,-1.02214689192185));
#112371=CARTESIAN_POINT('Ctrl Pts',(19.843175241912,17.4078214742779,-1.02086416357804));
#112372=CARTESIAN_POINT('Ctrl Pts',(19.8481018998733,17.4108612642901,-1.02051699468056));
#112373=CARTESIAN_POINT('Ctrl Pts',(19.8559115786694,17.4157242425549,-1.01996316173835));
#112374=CARTESIAN_POINT('Ctrl Pts',(19.8588028095931,17.4175342839147,-1.01975735882682));
#112375=CARTESIAN_POINT('Ctrl Pts',(19.8647626966768,17.4212855231065,-1.01933150900215));
#112376=CARTESIAN_POINT('Ctrl Pts',(19.8678307253766,17.4232276234367,-1.0191113991178));
#112377=CARTESIAN_POINT('Ctrl Pts',(19.8751293491352,17.4278740873608,-1.0185856696097));
#112378=CARTESIAN_POINT('Ctrl Pts',(19.879355333859,17.4305856185173,-1.01827957692072));
#112379=CARTESIAN_POINT('Ctrl Pts',(19.8935793862848,17.4397838398057,-1.01724370960489));
#112380=CARTESIAN_POINT('Ctrl Pts',(19.9035320997178,17.4463397800289,-1.01650952332952));
#112381=CARTESIAN_POINT('Ctrl Pts',(19.9273103183535,17.4622922153143,-1.0147338282345));
#112382=CARTESIAN_POINT('Ctrl Pts',(19.9410807314051,17.471768990872,-1.0136876733919));
#112383=CARTESIAN_POINT('Ctrl Pts',(19.9923045517757,17.5079224860696,-1.0097330682375));
#112384=CARTESIAN_POINT('Ctrl Pts',(20.0289959183228,17.5356527555774,-1.00677230862063));
#112385=CARTESIAN_POINT('Ctrl Pts',(20.1225742910843,17.6112881892137,-0.998935581656554));
#112386=CARTESIAN_POINT('Ctrl Pts',(20.177892152827,17.6610350522653,-0.994011792116405));
#112387=CARTESIAN_POINT('Ctrl Pts',(20.3402764466694,17.8233178585506,-0.97884485441687));
#112388=CARTESIAN_POINT('Ctrl Pts',(20.4376925012312,17.9448111597473,-0.968729204076044));
#112389=CARTESIAN_POINT('Ctrl Pts',(20.5337902901492,18.0960932858598,-0.957687396619167));
#112390=CARTESIAN_POINT('Ctrl Pts',(20.5462827913781,18.1165169130028,-0.956225130372346));
#112391=CARTESIAN_POINT('Ctrl Pts',(20.563346210817,18.1455069202426,-0.954188289951838));
#112392=CARTESIAN_POINT('Ctrl Pts',(20.5682083863896,18.1538989347082,-0.953603142493229));
#112393=CARTESIAN_POINT('Ctrl Pts',(20.5759803200287,18.1675282041206,-0.95265994467836));
#112394=CARTESIAN_POINT('Ctrl Pts',(20.5789257769284,18.1727448449722,-0.952300606916462));
#112395=CARTESIAN_POINT('Ctrl Pts',(20.5850180281273,18.1836424993465,-0.951553393936105));
#112396=CARTESIAN_POINT('Ctrl Pts',(20.5881609083949,18.1893256380664,-0.951165662243415));
#112397=CARTESIAN_POINT('Ctrl Pts',(20.5955277563842,18.202792758418,-0.950251396564215));
#112398=CARTESIAN_POINT('Ctrl Pts',(20.5997291506798,18.2105889996081,-0.949725672894765));
#112399=CARTESIAN_POINT('Ctrl Pts',(20.6135042310877,18.2365390965757,-0.947987338027659));
#112400=CARTESIAN_POINT('Ctrl Pts',(20.622863034932,18.2548061462338,-0.946782331584998));
#112401=CARTESIAN_POINT('Ctrl Pts',(20.671079376451,18.3523889117711,-0.940438849605809));
#112402=CARTESIAN_POINT('Ctrl Pts',(20.7052128150041,18.4339465173116,-0.935466838502114));
#112403=CARTESIAN_POINT('Ctrl Pts',(20.7770356875938,18.6410659637741,-0.923366564920433));
#112404=CARTESIAN_POINT('Ctrl Pts',(20.8083555698789,18.768431224881,-0.9163894775598));
#112405=CARTESIAN_POINT('Ctrl Pts',(20.8332930771479,18.9351735100264,-0.90708957052538));
#112406=CARTESIAN_POINT('Ctrl Pts',(20.8378739167237,18.972617979004,-0.904989142915688));
#112407=CARTESIAN_POINT('Ctrl Pts',(20.8458040228046,19.0558313986986,-0.900257365177248));
#112408=CARTESIAN_POINT('Ctrl Pts',(20.8486701978349,19.1016253978506,-0.897610763853716));
#112409=CARTESIAN_POINT('Ctrl Pts',(20.8502754963556,19.1550964974429,-0.894433888659794));
#112410=CARTESIAN_POINT('Ctrl Pts',(20.8504631740708,19.1627215689269,-0.893978808345923));
#112411=CARTESIAN_POINT('Ctrl Pts',(20.8506981096336,19.1749536612913,-0.893245243016827));
#112412=CARTESIAN_POINT('Ctrl Pts',(20.8507715425591,19.179560191593,-0.892968184348993));
#112413=CARTESIAN_POINT('Ctrl Pts',(20.8508753308635,19.1877479143726,-0.892474251672583));
#112414=CARTESIAN_POINT('Ctrl Pts',(20.8509116365179,19.1913289835225,-0.892257713650956));
#112415=CARTESIAN_POINT('Ctrl Pts',(20.8509695805185,19.1989526804795,-0.891795631580296));
#112416=CARTESIAN_POINT('Ctrl Pts',(20.8509887259094,19.2029952209265,-0.891549956635076));
#112417=CARTESIAN_POINT('Ctrl Pts',(20.8510092763564,19.2139751548644,-0.890880956095523));
#112418=CARTESIAN_POINT('Ctrl Pts',(20.8509881595329,19.2209124691406,-0.890456401210897));
#112419=CARTESIAN_POINT('Ctrl Pts',(20.8507068063256,19.2562611684461,-0.888284013714216));
#112420=CARTESIAN_POINT('Ctrl Pts',(20.8499087234104,19.2846638841337,-0.886508591043632));
#112421=CARTESIAN_POINT('Ctrl Pts',(20.8458846131126,19.3680539103531,-0.881224599527745));
#112422=CARTESIAN_POINT('Ctrl Pts',(20.8410840999099,19.4229394116035,-0.87765583949491));
#112423=CARTESIAN_POINT('Ctrl Pts',(20.8165298326325,19.6163873043886,-0.864885018400925));
#112424=CARTESIAN_POINT('Ctrl Pts',(20.7851878762934,19.7531278766494,-0.855533026123477));
#112425=CARTESIAN_POINT('Ctrl Pts',(20.7117632783027,19.9714705117818,-0.840658547782599));
#112426=CARTESIAN_POINT('Ctrl Pts',(20.6774831392652,20.0552393107478,-0.834959697909745));
#112427=CARTESIAN_POINT('Ctrl Pts',(20.6319419562892,20.1489199980843,-0.828603966027766));
#112428=CARTESIAN_POINT('Ctrl Pts',(20.6258176840833,20.1612123217394,-0.827770215727556));
#112429=CARTESIAN_POINT('Ctrl Pts',(20.6158033200141,20.1808319750147,-0.826439622383354));
#112430=CARTESIAN_POINT('Ctrl Pts',(20.6119890984143,20.1881973926852,-0.825940136924066));
#112431=CARTESIAN_POINT('Ctrl Pts',(20.60513933745,20.2012363246238,-0.825055898523691));
#112432=CARTESIAN_POINT('Ctrl Pts',(20.60212105194,20.2069187393921,-0.824670542748864));
#112433=CARTESIAN_POINT('Ctrl Pts',(20.5957778127672,20.2187306184847,-0.823869472659096));
#112434=CARTESIAN_POINT('Ctrl Pts',(20.5924483826109,20.2248576007023,-0.823453923214118));
#112435=CARTESIAN_POINT('Ctrl Pts',(20.583722144385,20.2407286327134,-0.822377375254052));
#112436=CARTESIAN_POINT('Ctrl Pts',(20.5782785544882,20.2504468187836,-0.82171805457273));
#112437=CARTESIAN_POINT('Ctrl Pts',(20.5542933360813,20.2924848601319,-0.818864949670978));
#112438=CARTESIAN_POINT('Ctrl Pts',(20.5349762899705,20.3243561804899,-0.816699232909909));
#112439=CARTESIAN_POINT('Ctrl Pts',(20.4814031028342,20.4077006157434,-0.811013082972562));
#112440=CARTESIAN_POINT('Ctrl Pts',(20.4457161800394,20.4582123094883,-0.807543793289486));
#112441=CARTESIAN_POINT('Ctrl Pts',(20.3211982712216,20.6190236951154,-0.79629125185731));
#112442=CARTESIAN_POINT('Ctrl Pts',(20.223525225247,20.7219736439583,-0.788766768521985));
#112443=CARTESIAN_POINT('Ctrl Pts',(20.0589248347197,20.8638775702418,-0.776736150204603));
#112444=CARTESIAN_POINT('Ctrl Pts',(19.9989286229428,20.9102301408278,-0.772455181743465));
#112445=CARTESIAN_POINT('Ctrl Pts',(19.9287599899443,20.958663574936,-0.767402204384557));
#112446=CARTESIAN_POINT('Ctrl Pts',(19.9208987847652,20.9640118858235,-0.766835470671899));
#112447=CARTESIAN_POINT('Ctrl Pts',(19.9091923300918,20.9718614443569,-0.765990165713417));
#112448=CARTESIAN_POINT('Ctrl Pts',(19.9053744241163,20.9744035262946,-0.765714268437201));
#112449=CARTESIAN_POINT('Ctrl Pts',(19.8985613494388,20.9789079968831,-0.76522149408285));
#112450=CARTESIAN_POINT('Ctrl Pts',(19.895569436007,20.9808752122895,-0.765004944767182));
#112451=CARTESIAN_POINT('Ctrl Pts',(19.889116818243,20.9850944687073,-0.764537580042762));
#112452=CARTESIAN_POINT('Ctrl Pts',(19.8856545563741,20.9873439503088,-0.764286605602603));
#112453=CARTESIAN_POINT('Ctrl Pts',(19.876070753523,20.9935308892412,-0.763591381927055));
#112454=CARTESIAN_POINT('Ctrl Pts',(19.8699355199932,20.9974468836334,-0.763145753095967));
#112455=CARTESIAN_POINT('Ctrl Pts',(19.8360559128462,21.0188264560479,-0.760682339576365));
#112456=CARTESIAN_POINT('Ctrl Pts',(19.8079305722278,21.035674377244,-0.75862785368423));
#112457=CARTESIAN_POINT('Ctrl Pts',(19.63711232465,21.1326822547788,-0.746145465528185));
#112458=CARTESIAN_POINT('Ctrl Pts',(19.4859092909409,21.1967258840482,-0.73512831277251));
#112459=CARTESIAN_POINT('Ctrl Pts',(19.2190444171249,21.2748578121306,-0.71698827893012));
#112460=CARTESIAN_POINT('Ctrl Pts',(19.1068117116188,21.2980543600943,-0.70970881956078));
#112461=CARTESIAN_POINT('Ctrl Pts',(18.9790781526786,21.3138145990478,-0.701850770658219));
#112462=CARTESIAN_POINT('Ctrl Pts',(18.9649012567325,21.3154184859781,-0.700984204352974));
#112463=CARTESIAN_POINT('Ctrl Pts',(18.9422949152857,21.3177448288807,-0.699611049189376));
#112464=CARTESIAN_POINT('Ctrl Pts',(18.9338756702896,21.3185602637674,-0.699101555770226));
#112465=CARTESIAN_POINT('Ctrl Pts',(18.9190081292988,21.319910347466,-0.698205143869056));
#112466=CARTESIAN_POINT('Ctrl Pts',(18.9125618877204,21.3204659312839,-0.697817573212883));
#112467=CARTESIAN_POINT('Ctrl Pts',(18.8992136022336,21.3215547578927,-0.697017252603145));
#112468=CARTESIAN_POINT('Ctrl Pts',(18.8923112791487,21.3220837172095,-0.69660464142529));
#112469=CARTESIAN_POINT('Ctrl Pts',(18.8745658310052,21.3233561181224,-0.695546938774859));
#112470=CARTESIAN_POINT('Ctrl Pts',(18.8637192659353,21.3240499381971,-0.69490340669241));
#112471=CARTESIAN_POINT('Ctrl Pts',(18.8182406329857,21.3266075582578,-0.692217108573733));
#112472=CARTESIAN_POINT('Ctrl Pts',(18.7835696213021,21.3277037771271,-0.69019837849321));
#112473=CARTESIAN_POINT('Ctrl Pts',(18.6930022215074,21.3283406221209,-0.684989114463495));
#112474=CARTESIAN_POINT('Ctrl Pts',(18.6371224591221,21.3265206306365,-0.681839180758607));
#112475=CARTESIAN_POINT('Ctrl Pts',(18.3834475168122,21.3081844708893,-0.667705160538776));
#112476=CARTESIAN_POINT('Ctrl Pts',(18.1885440302935,21.2661224211238,-0.657394732740525));
#112477=CARTESIAN_POINT('Ctrl Pts',(17.9724290328685,21.1865295053752,-0.644170670349927));
#112478=CARTESIAN_POINT('Ctrl Pts',(17.9427413969282,21.1748270650188,-0.642310098073312));
#112479=CARTESIAN_POINT('Ctrl Pts',(17.9070460265398,21.1598156963852,-0.640006153946296));
#112480=CARTESIAN_POINT('Ctrl Pts',(17.9007735587118,21.1571421292857,-0.639598759682576));
#112481=CARTESIAN_POINT('Ctrl Pts',(17.8904622900824,21.1526880834603,-0.63892468050851));
#112482=CARTESIAN_POINT('Ctrl Pts',(17.8864158931916,21.1509251693245,-0.638659042109389));
#112483=CARTESIAN_POINT('Ctrl Pts',(17.8791249403602,21.1477215172384,-0.638178342160083));
#112484=CARTESIAN_POINT('Ctrl Pts',(17.8758784656039,21.1462852593304,-0.637963556785933));
#112485=CARTESIAN_POINT('Ctrl Pts',(17.8695668896892,21.1434739798637,-0.637544520634806));
#112486=CARTESIAN_POINT('Ctrl Pts',(17.8665014919915,21.1420998480889,-0.637340332364547));
#112487=CARTESIAN_POINT('Ctrl Pts',(17.8574579143111,21.1380199874035,-0.636735977221489));
#112488=CARTESIAN_POINT('Ctrl Pts',(17.8514890956,21.1352937823569,-0.636334568963541));
#112489=CARTESIAN_POINT('Ctrl Pts',(17.8231334432058,21.1221829136873,-0.634415899126147));
#112490=CARTESIAN_POINT('Ctrl Pts',(17.8009176767315,21.1114355468693,-0.632877777299931));
#112491=CARTESIAN_POINT('Ctrl Pts',(17.738719949441,21.0799925751033,-0.628482634339698));
#112492=CARTESIAN_POINT('Ctrl Pts',(17.6992044461274,21.0584071729178,-0.625584854015875));
#112493=CARTESIAN_POINT('Ctrl Pts',(17.578480504402,20.9873727237562,-0.616463116042292));
#112494=CARTESIAN_POINT('Ctrl Pts',(17.4998930277222,20.9337027526604,-0.610137964857277));
#112495=CARTESIAN_POINT('Ctrl Pts',(17.3073680120026,20.7822661100353,-0.593981625990813));
#112496=CARTESIAN_POINT('Ctrl Pts',(17.1997115698409,20.6773325280377,-0.584307127283576));
#112497=CARTESIAN_POINT('Ctrl Pts',(17.0950142907436,20.5510054088362,-0.574290993645261));
#112498=CARTESIAN_POINT('Ctrl Pts',(17.0861068718918,20.5400360809597,-0.573432879666373));
#112499=CARTESIAN_POINT('Ctrl Pts',(17.0720937011992,20.5224216141066,-0.572073057614107));
#112500=CARTESIAN_POINT('Ctrl Pts',(17.0669165426599,20.515834068139,-0.571568473305881));
#112501=CARTESIAN_POINT('Ctrl Pts',(17.057848665583,20.5041538086771,-0.570680711877575));
#112502=CARTESIAN_POINT('Ctrl Pts',(17.0539417347495,20.4990738703728,-0.570296888909056));
#112503=CARTESIAN_POINT('Ctrl Pts',(17.0459029725944,20.4885227706918,-0.569504346541635));
#112504=CARTESIAN_POINT('Ctrl Pts',(17.0417745265418,20.4830491155068,-0.569095764192877));
#112505=CARTESIAN_POINT('Ctrl Pts',(17.0312342977279,20.4689323409043,-0.56804852865523));
#112506=CARTESIAN_POINT('Ctrl Pts',(17.0248616471264,20.4602601443962,-0.567411416658005));
#112507=CARTESIAN_POINT('Ctrl Pts',(16.9984537533301,20.4237427443155,-0.564754091846726));
#112508=CARTESIAN_POINT('Ctrl Pts',(16.9790300138077,20.3954603342814,-0.562757572607046));
#112509=CARTESIAN_POINT('Ctrl Pts',(16.9301570205903,20.3204541225425,-0.557608838260007));
#112510=CARTESIAN_POINT('Ctrl Pts',(16.9018328518384,20.2730273714807,-0.5544964948555));
#112511=CARTESIAN_POINT('Ctrl Pts',(16.8405517695375,20.1606520576168,-0.547383534944862));
#112512=CARTESIAN_POINT('Ctrl Pts',(16.809026302663,20.0950034808887,-0.543420741127947));
#112513=CARTESIAN_POINT('Ctrl Pts',(16.7673555757298,19.9953716183546,-0.537557186073658));
#112514=CARTESIAN_POINT('Ctrl Pts',(16.7545802484305,19.9625494382349,-0.535648358953803));
#112515=CARTESIAN_POINT('Ctrl Pts',(16.7287365187993,19.8909142528261,-0.531505687115641));
#112516=CARTESIAN_POINT('Ctrl Pts',(16.7159637149578,19.8520104643433,-0.529270377031467));
#112517=CARTESIAN_POINT('Ctrl Pts',(16.6989489234478,19.7946215484291,-0.52596417755349));
#112518=CARTESIAN_POINT('Ctrl Pts',(16.6938141846103,19.7764103006376,-0.524913722589127));
#112519=CARTESIAN_POINT('Ctrl Pts',(16.6732971358612,19.699721606859,-0.520475847901493));
#112520=CARTESIAN_POINT('Ctrl Pts',(16.660181126937,19.640673069453,-0.51702426761041));
#112521=CARTESIAN_POINT('Ctrl Pts',(16.6480273223415,19.5722326453611,-0.512901042489556));
#112522=CARTESIAN_POINT('Ctrl Pts',(16.6465009500222,19.5633049044344,-0.512360805496219));
#112523=CARTESIAN_POINT('Ctrl Pts',(16.644305604138,19.5499489430587,-0.511548681784569));
#112524=CARTESIAN_POINT('Ctrl Pts',(16.6435932942977,19.5455278134918,-0.511279208710169));
#112525=CARTESIAN_POINT('Ctrl Pts',(16.6423403665007,19.537590922247,-0.510794241488942));
#112526=CARTESIAN_POINT('Ctrl Pts',(16.6417945776022,19.5340760326778,-0.510579044653354));
#112527=CARTESIAN_POINT('Ctrl Pts',(16.640747943493,19.52722180465,-0.510158566898103));
#112528=CARTESIAN_POINT('Ctrl Pts',(16.640246230466,19.5238826521244,-0.509953342278624));
#112529=CARTESIAN_POINT('Ctrl Pts',(16.6391504869416,19.5164692620266,-0.509496889213461));
#112530=CARTESIAN_POINT('Ctrl Pts',(16.6385603510653,19.5123944747754,-0.509245445913275));
#112531=CARTESIAN_POINT('Ctrl Pts',(16.6371204772028,19.5022437235401,-0.508617740339853));
#112532=CARTESIAN_POINT('Ctrl Pts',(16.6362852638928,19.4961657824301,-0.508240703202683));
#112533=CARTESIAN_POINT('Ctrl Pts',(16.6323977852852,19.4669346043774,-0.50642195905365));
#112534=CARTESIAN_POINT('Ctrl Pts',(16.6297024930675,19.4437365273374,-0.504962251941544));
#112535=CARTESIAN_POINT('Ctrl Pts',(16.6205187012968,19.351389617802,-0.499098993300709));
#112536=CARTESIAN_POINT('Ctrl Pts',(16.6170514727118,19.2819895701451,-0.494577329568077));
#112537=CARTESIAN_POINT('Ctrl Pts',(16.617000568856,19.2125519458626,-0.490010468414517));
#112538=CARTESIAN_POINT('Ctrl Pts',(16.617000615792,19.2126147021618,-0.489056278967189));
#112539=CARTESIAN_POINT('Ctrl Pts',(16.6169459704489,19.1409704320946,-0.484732818395265));
#112540=CARTESIAN_POINT('Ctrl Pts',(16.6205324586778,19.0691916432072,-0.480409357823342));
#112541=CARTESIAN_POINT('Ctrl Pts',(16.6277745421012,18.9976849266948,-0.476085897251419));
#112542=CARTESIAN_POINT('Ctrl Pts',(16.6350090269828,18.9262532364906,-0.471766972942677));
#112543=CARTESIAN_POINT('Ctrl Pts',(16.645891455306,18.8550935436973,-0.467448048633935));
#112544=CARTESIAN_POINT('Ctrl Pts',(16.6603842665429,18.7846119256369,-0.463129124325193));
#112545=CARTESIAN_POINT('Ctrl Pts',(16.6748666504054,18.714181018112,-0.4588133074219));
#112546=CARTESIAN_POINT('Ctrl Pts',(16.6929541651129,18.6444277026836,-0.454497490518607));
#112547=CARTESIAN_POINT('Ctrl Pts',(16.7145577237428,18.5757505270643,-0.450181673615314));
#112548=CARTESIAN_POINT('Ctrl Pts',(16.7241553570749,18.545239889388,-0.448264321531073));
#112549=CARTESIAN_POINT('Ctrl Pts',(16.7344462704266,18.5149415151545,-0.446346969446833));
#112550=CARTESIAN_POINT('Ctrl Pts',(16.7454194503191,18.4848895418526,-0.444429617362593));
#112551=CARTESIAN_POINT('Origin',(18.734,-18.952,0.));
#112552=CARTESIAN_POINT('',(16.6170002905271,-18.9508909049916,-0.710943720977502));
#112553=CARTESIAN_POINT('Ctrl Pts',(16.7454194499637,-19.6781104571739,
-0.666446448202515));
#112554=CARTESIAN_POINT('Ctrl Pts',(16.7201110311403,-19.6087989234712,
-0.670880799931208));
#112555=CARTESIAN_POINT('Ctrl Pts',(16.6984028489342,-19.5380871560008,
-0.675315151659902));
#112556=CARTESIAN_POINT('Ctrl Pts',(16.6804409278771,-19.4663774268974,
-0.679749503388595));
#112557=CARTESIAN_POINT('Ctrl Pts',(16.6624933915782,-19.3947251263463,
-0.684180303878107));
#112558=CARTESIAN_POINT('Ctrl Pts',(16.6482862689509,-19.3220769011711,
-0.688611104367619));
#112559=CARTESIAN_POINT('Ctrl Pts',(16.6379158183503,-19.2488503047633,
-0.693041904857131));
#112560=CARTESIAN_POINT('Ctrl Pts',(16.6275504654133,-19.1756597033728,
-0.697470527357381));
#112561=CARTESIAN_POINT('Ctrl Pts',(16.6210181017774,-19.1018917551645,
-0.701899149857632));
#112562=CARTESIAN_POINT('Ctrl Pts',(16.6183636617623,-19.0279729183858,
-0.706327772357882));
#112563=CARTESIAN_POINT('Ctrl Pts',(16.6174414217412,-19.0022910761897,
-0.707866421897756));
#112564=CARTESIAN_POINT('Ctrl Pts',(16.6169868262232,-18.976591072574,-0.709405071437629));
#112565=CARTESIAN_POINT('Ctrl Pts',(16.6170002905271,-18.9508909049916,
-0.710943720977502));
#112566=CARTESIAN_POINT('Ctrl Pts',(16.6170002428037,-18.9509860813785,
-0.71261911997228));
#112567=CARTESIAN_POINT('Ctrl Pts',(16.6170355426432,-18.8772821863969,
-0.71680613931656));
#112568=CARTESIAN_POINT('Ctrl Pts',(16.6209198238468,-18.8036252920842,
-0.720887471493913));
#112569=CARTESIAN_POINT('Ctrl Pts',(16.6457836173313,-18.5674910391913,
-0.733880950583028));
#112570=CARTESIAN_POINT('Ctrl Pts',(16.6817565015368,-18.4072256903138,
-0.742529972060711));
#112571=CARTESIAN_POINT('Ctrl Pts',(16.7460896191493,-18.2233937368426,
-0.753730253773707));
#112572=CARTESIAN_POINT('Ctrl Pts',(16.7569987507012,-18.1942925374262,
-0.755544779403702));
#112573=CARTESIAN_POINT('Ctrl Pts',(16.7711944231595,-18.1588202190053,
-0.757820171089045));
#112574=CARTESIAN_POINT('Ctrl Pts',(16.7738785229288,-18.1522102218227,
-0.75824692452464));
#112575=CARTESIAN_POINT('Ctrl Pts',(16.7781515132025,-18.1418380566543,
-0.758921095400191));
#112576=CARTESIAN_POINT('Ctrl Pts',(16.7797179957211,-18.1380666336509,
-0.75916717565633));
#112577=CARTESIAN_POINT('Ctrl Pts',(16.7826759254017,-18.1310029653032,
-0.759629887068448));
#112578=CARTESIAN_POINT('Ctrl Pts',(16.7840648014493,-18.1277097017187,
-0.759846361949575));
#112579=CARTESIAN_POINT('Ctrl Pts',(16.7872660989969,-18.1201722433198,
-0.760343519957725));
#112580=CARTESIAN_POINT('Ctrl Pts',(16.7890840600327,-18.1159304552678,
-0.7606245371859));
#112581=CARTESIAN_POINT('Ctrl Pts',(16.7947542407714,-18.102818984733,-0.761496922286903));
#112582=CARTESIAN_POINT('Ctrl Pts',(16.7986533115283,-18.0939698731072,
-0.762091039278325));
#112583=CARTESIAN_POINT('Ctrl Pts',(16.8403369192543,-18.00109682771,-0.768380309550798));
#112584=CARTESIAN_POINT('Ctrl Pts',(16.8835033415036,-17.9196072284535,
-0.774361178149046));
#112585=CARTESIAN_POINT('Ctrl Pts',(16.9959657519195,-17.7371479806969,
-0.788456678379995));
#112586=CARTESIAN_POINT('Ctrl Pts',(17.0689947662275,-17.6388399003217,
-0.796593907650438));
#112587=CARTESIAN_POINT('Ctrl Pts',(17.1923918239987,-17.4996928903399,
-0.808626273526529));
#112588=CARTESIAN_POINT('Ctrl Pts',(17.2368175647855,-17.453935350144,-0.812685605840463));
#112589=CARTESIAN_POINT('Ctrl Pts',(17.3015997566456,-17.3929766520606,
-0.818232054003031));
#112590=CARTESIAN_POINT('Ctrl Pts',(17.3202629042825,-17.3760330695435,
-0.81979016167976));
#112591=CARTESIAN_POINT('Ctrl Pts',(17.3490355213559,-17.3508340284309,
-0.82213340014388));
#112592=CARTESIAN_POINT('Ctrl Pts',(17.3589255684514,-17.3423325202814,
-0.822928630515614));
#112593=CARTESIAN_POINT('Ctrl Pts',(17.3772963109687,-17.326833868013,-0.82438726746762));
#112594=CARTESIAN_POINT('Ctrl Pts',(17.3857541133686,-17.3198103992765,
-0.825051739970025));
#112595=CARTESIAN_POINT('Ctrl Pts',(17.3995560471391,-17.3085295836163,
-0.826124784077197));
#112596=CARTESIAN_POINT('Ctrl Pts',(17.4048666696862,-17.3042317320671,
-0.826534994193013));
#112597=CARTESIAN_POINT('Ctrl Pts',(17.4149606219979,-17.2961433136996,
-0.827309690418029));
#112598=CARTESIAN_POINT('Ctrl Pts',(17.4197397094547,-17.2923475857319,
-0.827674381729845));
#112599=CARTESIAN_POINT('Ctrl Pts',(17.4308937937994,-17.2835669917952,
-0.828520726216034));
#112600=CARTESIAN_POINT('Ctrl Pts',(17.4372811196317,-17.2785978858684,
-0.82900174839417));
#112601=CARTESIAN_POINT('Ctrl Pts',(17.4538175285942,-17.2658846989307,
-0.830237875951687));
#112602=CARTESIAN_POINT('Ctrl Pts',(17.4640085401947,-17.2581955038162,
-0.830990818829536));
#112603=CARTESIAN_POINT('Ctrl Pts',(17.5289624618929,-17.2101030885643,
-0.835735356583544));
#112604=CARTESIAN_POINT('Ctrl Pts',(17.5855804178744,-17.1722657100199,
-0.839626364752976));
#112605=CARTESIAN_POINT('Ctrl Pts',(17.7838167681934,-17.0531924166677,
-0.852592511231799));
#112606=CARTESIAN_POINT('Ctrl Pts',(17.9329436580573,-16.9856264318967,
-0.861226753026156));
#112607=CARTESIAN_POINT('Ctrl Pts',(18.1411303138149,-16.9189564153889,
-0.873301274503703));
#112608=CARTESIAN_POINT('Ctrl Pts',(18.1945524665604,-16.9041337479739,
-0.876406525842522));
#112609=CARTESIAN_POINT('Ctrl Pts',(18.2762612297136,-16.884881656752,-0.881248542072119));
#112610=CARTESIAN_POINT('Ctrl Pts',(18.3041598476546,-16.8789008008341,
-0.882917908553437));
#112611=CARTESIAN_POINT('Ctrl Pts',(18.3389930273685,-16.8721666421691,
-0.885031716162564));
#112612=CARTESIAN_POINT('Ctrl Pts',(18.3458231882031,-16.8708810546962,
-0.885447598510661));
#112613=CARTESIAN_POINT('Ctrl Pts',(18.3566405913668,-16.8689000845491,
-0.886108654377235));
#112614=CARTESIAN_POINT('Ctrl Pts',(18.3606237796473,-16.8681824507699,
-0.886352581239698));
#112615=CARTESIAN_POINT('Ctrl Pts',(18.3681384624805,-16.8668508005615,
-0.886813781301725));
#112616=CARTESIAN_POINT('Ctrl Pts',(18.3716694666074,-16.8662343294563,
-0.887030913233596));
#112617=CARTESIAN_POINT('Ctrl Pts',(18.3797450055537,-16.8648455619696,
-0.887528456116828));
#112618=CARTESIAN_POINT('Ctrl Pts',(18.3842905010985,-16.8640791406926,
-0.887809196000663));
#112619=CARTESIAN_POINT('Ctrl Pts',(18.3963642288273,-16.8620839082306,
-0.888556652553524));
#112620=CARTESIAN_POINT('Ctrl Pts',(18.4038965813485,-16.8608809422738,
-0.889024773657226));
#112621=CARTESIAN_POINT('Ctrl Pts',(18.4566786031498,-16.8527435920211,
-0.892316956169591));
#112622=CARTESIAN_POINT('Ctrl Pts',(18.5021328400444,-16.8472383611177,
-0.895212973041072));
#112623=CARTESIAN_POINT('Ctrl Pts',(18.551351529235,-16.8428907603699,-0.898389467614695));
#112624=CARTESIAN_POINT('Ctrl Pts',(18.5549780714355,-16.8425798433235,
-0.8986237573938));
#112625=CARTESIAN_POINT('Ctrl Pts',(18.565504661746,-16.841704700739,-0.899304479954829));
#112626=CARTESIAN_POINT('Ctrl Pts',(18.572406655665,-16.8411649712813,-0.89975163445017));
#112627=CARTESIAN_POINT('Ctrl Pts',(18.7317404347313,-16.8294912688356,
-0.910091580626856));
#112628=CARTESIAN_POINT('Ctrl Pts',(18.8849319967157,-16.8348623850344,
-0.920355985649072));
#112629=CARTESIAN_POINT('Ctrl Pts',(19.1280890125997,-16.869933960768,-0.936300890317911));
#112630=CARTESIAN_POINT('Ctrl Pts',(19.2189995374875,-16.8892143769221,
-0.942191256988144));
#112631=CARTESIAN_POINT('Ctrl Pts',(19.3286545583813,-16.9201241464266,
-0.949187184418303));
#112632=CARTESIAN_POINT('Ctrl Pts',(19.3488615490117,-16.9261473760029,
-0.950472061642716));
#112633=CARTESIAN_POINT('Ctrl Pts',(19.3775210786797,-16.9351584439184,
-0.952288796585128));
#112634=CARTESIAN_POINT('Ctrl Pts',(19.3860493412802,-16.937899480802,-0.952828694998408));
#112635=CARTESIAN_POINT('Ctrl Pts',(19.4007517722814,-16.9427281053334,
-0.953758306041049));
#112636=CARTESIAN_POINT('Ctrl Pts',(19.4069341214739,-16.944790209727,-0.954148851503725));
#112637=CARTESIAN_POINT('Ctrl Pts',(19.4187670220499,-16.948797854094,-0.95489570394616));
#112638=CARTESIAN_POINT('Ctrl Pts',(19.4244190418326,-16.9507388327227,
-0.955252157219276));
#112639=CARTESIAN_POINT('Ctrl Pts',(19.4391249210422,-16.9558587420666,
-0.956178909538389));
#112640=CARTESIAN_POINT('Ctrl Pts',(19.4481655852883,-16.9590753658766,
-0.956747954111838));
#112641=CARTESIAN_POINT('Ctrl Pts',(19.479073034196,-16.970309410156,-0.95869123758568));
#112642=CARTESIAN_POINT('Ctrl Pts',(19.5008297091688,-16.9786263200856,
-0.96005550196899));
#112643=CARTESIAN_POINT('Ctrl Pts',(19.681256356536,-17.0510325973115,-0.971349221504955));
#112644=CARTESIAN_POINT('Ctrl Pts',(19.8317541182695,-17.1337826213133,
-0.980570505987134));
#112645=CARTESIAN_POINT('Ctrl Pts',(20.0438142572456,-17.2864072233282,
-0.994777264474122));
#112646=CARTESIAN_POINT('Ctrl Pts',(20.1135259674386,-17.3436722316453,
-0.999701756439865));
#112647=CARTESIAN_POINT('Ctrl Pts',(20.2075773503907,-17.4315562820003,
-1.00704518389461));
#112648=CARTESIAN_POINT('Ctrl Pts',(20.2350557938208,-17.4586780694052,
-1.00928629483316));
#112649=CARTESIAN_POINT('Ctrl Pts',(20.2670471553504,-17.4920296529738,
-1.01203567545134));
#112650=CARTESIAN_POINT('Ctrl Pts',(20.2722890530305,-17.4975537892179,
-1.01249085978528));
#112651=CARTESIAN_POINT('Ctrl Pts',(20.2803696947564,-17.5061620642462,
-1.01320008634213));
#112652=CARTESIAN_POINT('Ctrl Pts',(20.2832293374995,-17.509226619161,-1.0134525545708));
#112653=CARTESIAN_POINT('Ctrl Pts',(20.2885026678211,-17.5149115725923,
-1.01392091358897));
#112654=CARTESIAN_POINT('Ctrl Pts',(20.290918849221,-17.5175295789655,-1.0141366090273));
#112655=CARTESIAN_POINT('Ctrl Pts',(20.2963498247981,-17.5234440925452,
-1.01462391795212));
#112656=CARTESIAN_POINT('Ctrl Pts',(20.2993607813639,-17.5267440303257,
-1.01489581413903));
#112657=CARTESIAN_POINT('Ctrl Pts',(20.3081694998761,-17.5364597630036,
-1.01569629102243));
#112658=CARTESIAN_POINT('Ctrl Pts',(20.3139383412456,-17.5429014907017,
-1.01622696668769));
#112659=CARTESIAN_POINT('Ctrl Pts',(20.3539119531124,-17.5880917602718,
-1.01994825404022));
#112660=CARTESIAN_POINT('Ctrl Pts',(20.3867242811015,-17.6280430822312,
-1.02323002510233));
#112661=CARTESIAN_POINT('Ctrl Pts',(20.4313955828887,-17.6866845998212,
-1.02798917296889));
#112662=CARTESIAN_POINT('Ctrl Pts',(20.4444772056338,-17.7044253494656,
-1.02942182313896));
#112663=CARTESIAN_POINT('Ctrl Pts',(20.4839575658919,-17.7597554046055,
-1.03386120766503));
#112664=CARTESIAN_POINT('Ctrl Pts',(20.5094115651562,-17.7980016302671,
-1.03688954573458));
#112665=CARTESIAN_POINT('Ctrl Pts',(20.5911954782104,-17.9300054568297,
-1.04714745521377));
#112666=CARTESIAN_POINT('Ctrl Pts',(20.6415049546145,-18.0272966930861,
-1.05437844370008));
#112667=CARTESIAN_POINT('Ctrl Pts',(20.7055081741047,-18.1787746546412,
-1.06494831847687));
#112668=CARTESIAN_POINT('Ctrl Pts',(20.7249562726974,-18.2303242726602,
-1.06843561308593));
#112669=CARTESIAN_POINT('Ctrl Pts',(20.7532158627143,-18.3151074879787,
-1.07399052678027));
#112670=CARTESIAN_POINT('Ctrl Pts',(20.763267171779,-18.3478975800922,-1.07609654636897));
#112671=CARTESIAN_POINT('Ctrl Pts',(20.7754329830177,-18.391324384167,-1.07883209796092));
#112672=CARTESIAN_POINT('Ctrl Pts',(20.7782683421713,-18.4017521264737,
-1.07948495512259));
#112673=CARTESIAN_POINT('Ctrl Pts',(20.7827823701362,-18.418870215392,-1.08055024085139));
#112674=CARTESIAN_POINT('Ctrl Pts',(20.7845083805336,-18.425547769945,-1.08096419825283));
#112675=CARTESIAN_POINT('Ctrl Pts',(20.7877868246637,-18.4384921043285,
-1.08176360147426));
#112676=CARTESIAN_POINT('Ctrl Pts',(20.7893432824945,-18.4447577771819,
-1.08214917352929));
#112677=CARTESIAN_POINT('Ctrl Pts',(20.7928716566639,-18.4592445096494,
-1.08303751570866));
#112678=CARTESIAN_POINT('Ctrl Pts',(20.7948230470711,-18.4674704924275,
-1.08353961967391));
#112679=CARTESIAN_POINT('Ctrl Pts',(20.7999401120983,-18.4896314765021,
-1.08488619381826));
#112680=CARTESIAN_POINT('Ctrl Pts',(20.8030140925656,-18.5035873574756,
-1.08572772199579));
#112681=CARTESIAN_POINT('Ctrl Pts',(20.8299391651873,-18.6320033708402,
-1.09341430053484));
#112682=CARTESIAN_POINT('Ctrl Pts',(20.8444128240033,-18.7482309858231,
-1.0999421474991));
#112683=CARTESIAN_POINT('Ctrl Pts',(20.8559026254581,-19.0278147569397,
-1.11526007103807));
#112684=CARTESIAN_POINT('Ctrl Pts',(20.8437863098804,-19.1907643877648,
-1.12386688060966));
#112685=CARTESIAN_POINT('Ctrl Pts',(20.8070320242304,-19.3824319035813,
-1.13507492961851));
#112686=CARTESIAN_POINT('Ctrl Pts',(20.800220164733,-19.4140252925404,-1.13696008886946));
#112687=CARTESIAN_POINT('Ctrl Pts',(20.7910040714245,-19.4524752374912,
-1.13931434469167));
#112688=CARTESIAN_POINT('Ctrl Pts',(20.7892838660647,-19.4594932902695,
-1.13974651843837));
#112689=CARTESIAN_POINT('Ctrl Pts',(20.7865298132606,-19.4704855135526,
-1.14042748937319));
#112690=CARTESIAN_POINT('Ctrl Pts',(20.7855202550648,-19.4744657926485,
-1.14067490717982));
#112691=CARTESIAN_POINT('Ctrl Pts',(20.7836108095494,-19.4819030951674,
-1.14113882890266));
#112692=CARTESIAN_POINT('Ctrl Pts',(20.7827137504395,-19.4853607868861,
-1.14135516863377));
#112693=CARTESIAN_POINT('Ctrl Pts',(20.7806450938112,-19.4932521501384,
-1.14185040478401));
#112694=CARTESIAN_POINT('Ctrl Pts',(20.7794678424307,-19.4976842811726,
-1.14212962465978));
#112695=CARTESIAN_POINT('Ctrl Pts',(20.7758018608328,-19.5113074562963,
-1.1429911020694));
#112696=CARTESIAN_POINT('Ctrl Pts',(20.7732655530011,-19.5204854141741,
-1.14357601276167));
#112697=CARTESIAN_POINT('Ctrl Pts',(20.7494657818614,-19.6043988155693,
-1.14896340429626));
#112698=CARTESIAN_POINT('Ctrl Pts',(20.7241668174136,-19.6779200213361,
-1.15397020109261));
#112699=CARTESIAN_POINT('Ctrl Pts',(20.6794746347646,-19.7877571648899,
-1.16173136192276));
#112700=CARTESIAN_POINT('Ctrl Pts',(20.6629666402308,-19.8251833525167,
-1.16442845492379));
#112701=CARTESIAN_POINT('Ctrl Pts',(20.5983938185803,-19.9607976586218,
-1.1743505843766));
#112702=CARTESIAN_POINT('Ctrl Pts',(20.5438256082449,-20.0557081870924,
-1.18157789139431));
#112703=CARTESIAN_POINT('Ctrl Pts',(20.4511414131881,-20.1914113959507,
-1.1921400866996));
#112704=CARTESIAN_POINT('Ctrl Pts',(20.4183544039852,-20.2356145450826,
-1.19562338255792));
#112705=CARTESIAN_POINT('Ctrl Pts',(20.362410968956,-20.3051964763336,-1.20117277541098));
#112706=CARTESIAN_POINT('Ctrl Pts',(20.3402957383787,-20.3313756572483,
-1.20327716706276));
#112707=CARTESIAN_POINT('Ctrl Pts',(20.3103831203905,-20.3650895196156,
-1.20601102786557));
#112708=CARTESIAN_POINT('Ctrl Pts',(20.3031506775416,-20.3731164240299,
-1.20666377933687));
#112709=CARTESIAN_POINT('Ctrl Pts',(20.2912008945218,-20.3861764005765,
-1.20772898915887));
#112710=CARTESIAN_POINT('Ctrl Pts',(20.2865199113978,-20.3912423355137,
-1.20814297506961));
#112711=CARTESIAN_POINT('Ctrl Pts',(20.2774086500694,-20.4010067077372,
-1.20894250056905));
#112712=CARTESIAN_POINT('Ctrl Pts',(20.272981473681,-20.4057079229574,-1.20932816606182));
#112713=CARTESIAN_POINT('Ctrl Pts',(20.2627063105642,-20.4165195628214,
-1.21021682030486));
#112714=CARTESIAN_POINT('Ctrl Pts',(20.2568430529755,-20.4226153722222,
-1.21071914209565));
#112715=CARTESIAN_POINT('Ctrl Pts',(20.240968867543,-20.4389224300737,-1.21206651788627));
#112716=CARTESIAN_POINT('Ctrl Pts',(20.230890641896,-20.4490677679866,-1.21290862561043));
#112717=CARTESIAN_POINT('Ctrl Pts',(20.1369967599727,-20.5416907055649,
-1.22063511917889));
#112718=CARTESIAN_POINT('Ctrl Pts',(20.0465436656997,-20.6171579230743,
-1.22719842020855));
#112719=CARTESIAN_POINT('Ctrl Pts',(19.8163414313007,-20.7787470044817,
-1.24259189043989));
#112720=CARTESIAN_POINT('Ctrl Pts',(19.6719713496131,-20.8569055057939,
-1.2512387110801));
#112721=CARTESIAN_POINT('Ctrl Pts',(19.4912802367099,-20.9291637818119,
-1.26243141537735));
#112722=CARTESIAN_POINT('Ctrl Pts',(19.462249148109,-20.94003997112,-1.26424161042471));
#112723=CARTESIAN_POINT('Ctrl Pts',(19.4262575060555,-20.9526297610663,
-1.26651245160639));
#112724=CARTESIAN_POINT('Ctrl Pts',(19.4195117350713,-20.9549512109224,
-1.26693920475872));
#112725=CARTESIAN_POINT('Ctrl Pts',(19.4088835218168,-20.958548761691,-1.26761354742592));
#112726=CARTESIAN_POINT('Ctrl Pts',(19.4050088263892,-20.9598478167734,
-1.26785980230966));
#112727=CARTESIAN_POINT('Ctrl Pts',(19.3977369032497,-20.9622624477946,
-1.26832278072534));
#112728=CARTESIAN_POINT('Ctrl Pts',(19.3943406024634,-20.963380638718,-1.26853934755794));
#112729=CARTESIAN_POINT('Ctrl Pts',(19.3865516696503,-20.9659231967643,
-1.26903677178193));
#112730=CARTESIAN_POINT('Ctrl Pts',(19.3821572121935,-20.9673417951746,
-1.26931796337629));
#112731=CARTESIAN_POINT('Ctrl Pts',(19.3685310772336,-20.9716913444586,
-1.27019148941984));
#112732=CARTESIAN_POINT('Ctrl Pts',(19.3592840523413,-20.9745732769327,
-1.27078658354604));
#112733=CARTESIAN_POINT('Ctrl Pts',(19.2480925145358,-21.0083919047543,
-1.27796710962819));
#112734=CARTESIAN_POINT('Ctrl Pts',(19.1439841050508,-21.0316505536747,
-1.28493246285752));
#112735=CARTESIAN_POINT('Ctrl Pts',(18.9302683587808,-21.0627220560751,
-1.29917889280898));
#112736=CARTESIAN_POINT('Ctrl Pts',(18.8208889906715,-21.0700467351152,
-1.30643960358215));
#112737=CARTESIAN_POINT('Ctrl Pts',(18.6488176405106,-21.0682121108594,
-1.31756396746955));
#112738=CARTESIAN_POINT('Ctrl Pts',(18.5862617189313,-21.0647669783043,
-1.32154889443608));
#112739=CARTESIAN_POINT('Ctrl Pts',(18.4991729974121,-21.0560829510683,
-1.32700390567964));
#112740=CARTESIAN_POINT('Ctrl Pts',(18.4744450717296,-21.053175886837,-1.32854246750262));
#112741=CARTESIAN_POINT('Ctrl Pts',(18.4312398161399,-21.0473221870459,
-1.33121312181506));
#112742=CARTESIAN_POINT('Ctrl Pts',(18.4127399434587,-21.0445656041731,
-1.3323509954114));
#112743=CARTESIAN_POINT('Ctrl Pts',(18.3858541383861,-21.04019450859,-1.33399683591618));
#112744=CARTESIAN_POINT('Ctrl Pts',(18.3774379901541,-21.0387739175895,
-1.3345109188948));
#112745=CARTESIAN_POINT('Ctrl Pts',(18.3626808477277,-21.0361911239433,
-1.33541042756147));
#112746=CARTESIAN_POINT('Ctrl Pts',(18.3563361850225,-21.0350507910876,
-1.33579654268471));
#112747=CARTESIAN_POINT('Ctrl Pts',(18.3440143891395,-21.0327780347425,
-1.33654523976477));
#112748=CARTESIAN_POINT('Ctrl Pts',(18.3380367400237,-21.0316487935424,
-1.33690791883884));
#112749=CARTESIAN_POINT('Ctrl Pts',(18.3237391321155,-21.0288839436055,
-1.33777415045736));
#112750=CARTESIAN_POINT('Ctrl Pts',(18.3154239278694,-21.0272240770436,
-1.33827692584218));
#112751=CARTESIAN_POINT('Ctrl Pts',(18.2853391240321,-21.0210304199913,
-1.34009252277639));
#112752=CARTESIAN_POINT('Ctrl Pts',(18.2636308422363,-21.0162035682387,
-1.34139599073438));
#112753=CARTESIAN_POINT('Ctrl Pts',(18.0627496913366,-20.9682038497831,
-1.35340658175214));
#112754=CARTESIAN_POINT('Ctrl Pts',(17.8898620219208,-20.9021518255334,
-1.36327111787147));
#112755=CARTESIAN_POINT('Ctrl Pts',(17.6564395998259,-20.7760376059843,
-1.3777304261534));
#112756=CARTESIAN_POINT('Ctrl Pts',(17.5874515606887,-20.7334809082973,
-1.38218217778131));
#112757=CARTESIAN_POINT('Ctrl Pts',(17.4913584157976,-20.6663061783925,
-1.38888706854443));
#112758=CARTESIAN_POINT('Ctrl Pts',(17.4621806469295,-20.6447725654575,
-1.39099580212177));
#112759=CARTESIAN_POINT('Ctrl Pts',(17.4276698019771,-20.6179070696227,
-1.39359844041197));
#112760=CARTESIAN_POINT('Ctrl Pts',(17.4217918827532,-20.6132810731869,
-1.39404562883981));
#112761=CARTESIAN_POINT('Ctrl Pts',(17.4126815718345,-20.606032628465,-1.39474505449033));
#112762=CARTESIAN_POINT('Ctrl Pts',(17.4094321231862,-20.6034315800736,
-1.39499578678139));
#112763=CARTESIAN_POINT('Ctrl Pts',(17.4034133841137,-20.5985846381858,
-1.39546259551572));
#112764=CARTESIAN_POINT('Ctrl Pts',(17.4006420892115,-20.5963413253399,
-1.39567848727596));
#112765=CARTESIAN_POINT('Ctrl Pts',(17.394381034439,-20.5912468802355,-1.39616839597726));
#112766=CARTESIAN_POINT('Ctrl Pts',(17.3908947210674,-20.588391614525,-1.39644270902803));
#112767=CARTESIAN_POINT('Ctrl Pts',(17.3806055911754,-20.5799098593907,
-1.39725672607667));
#112768=CARTESIAN_POINT('Ctrl Pts',(17.3738289215356,-20.5742520048436,
-1.39779863000167));
#112769=CARTESIAN_POINT('Ctrl Pts',(17.3242110073926,-20.5322964589429,
-1.40180781333197));
#112770=CARTESIAN_POINT('Ctrl Pts',(17.282797325454,-20.4943525903393,-1.40538257912108));
#112771=CARTESIAN_POINT('Ctrl Pts',(17.1985944106414,-20.4108083883091,
-1.41306225783972));
#112772=CARTESIAN_POINT('Ctrl Pts',(17.1562154909218,-20.3648650558648,
-1.41717756742601));
#112773=CARTESIAN_POINT('Ctrl Pts',(17.0452481667157,-20.23333592099,-1.42854452694169));
#112774=CARTESIAN_POINT('Ctrl Pts',(16.9811727592963,-20.1441848096651,
-1.43579413788716));
#112775=CARTESIAN_POINT('Ctrl Pts',(16.8955511281902,-20.0031241016455,
-1.44640313660375));
#112776=CARTESIAN_POINT('Ctrl Pts',(16.8686817957824,-19.9546689190305,
-1.44991078270719));
#112777=CARTESIAN_POINT('Ctrl Pts',(16.8282391775142,-19.874469582801,-1.45549436127309));
#112778=CARTESIAN_POINT('Ctrl Pts',(16.8134880371499,-19.8433520421174,
-1.4576091835182));
#112779=CARTESIAN_POINT('Ctrl Pts',(16.795105725082,-19.8019971329562,-1.46035436886814));
#112780=CARTESIAN_POINT('Ctrl Pts',(16.7907854995237,-19.7920735368376,
-1.46100825898826));
#112781=CARTESIAN_POINT('Ctrl Pts',(16.7838354397002,-19.7757686648256,
-1.46207482888022));
#112782=CARTESIAN_POINT('Ctrl Pts',(16.7811604113993,-19.7694069784057,
-1.46248904410319));
#112783=CARTESIAN_POINT('Ctrl Pts',(16.7760434438126,-19.7570694352098,
-1.46328866860384));
#112784=CARTESIAN_POINT('Ctrl Pts',(16.7735976392193,-19.7510952738546,
-1.46367420557897));
#112785=CARTESIAN_POINT('Ctrl Pts',(16.7680147558737,-19.7372785269574,
-1.46456207246422));
#112786=CARTESIAN_POINT('Ctrl Pts',(16.7648971978317,-19.7294281334439,
-1.46506373891318));
#112787=CARTESIAN_POINT('Ctrl Pts',(16.7566421296176,-19.7082726131605,
-1.4664082666197));
#112788=CARTESIAN_POINT('Ctrl Pts',(16.7515918954761,-19.6949337352172,
-1.46724820074698));
#112789=CARTESIAN_POINT('Ctrl Pts',(16.7462566539521,-19.6804002171314,
-1.4681552115446));
#112790=CARTESIAN_POINT('Ctrl Pts',(16.745837552997,-19.6792555054942,-1.46822659633938));
#112791=CARTESIAN_POINT('Ctrl Pts',(16.7454194501222,-19.6781104576079,
-1.46829794770746));
#112792=CARTESIAN_POINT('',(16.6170006157907,-18.95038529957,-0.489056278967188));
#112793=CARTESIAN_POINT('Ctrl Pts',(16.7454193881274,-19.6781102878244,
-1.24458621709267));
#112794=CARTESIAN_POINT('Ctrl Pts',(16.8018177033943,-19.832566984228,-1.23372059953188));
#112795=CARTESIAN_POINT('Ctrl Pts',(16.8760653146766,-19.9800494973809,
-1.22298084368604));
#112796=CARTESIAN_POINT('Ctrl Pts',(16.9785115316654,-20.1353880728159,
-1.21154550124883));
#112797=CARTESIAN_POINT('Ctrl Pts',(16.9905656874721,-20.1530761607974,
-1.21024028032419));
#112798=CARTESIAN_POINT('Ctrl Pts',(17.0076902625298,-20.1774033377812,
-1.20844022578061));
#112799=CARTESIAN_POINT('Ctrl Pts',(17.0125345191703,-20.1841993553649,
-1.20793681684617));
#112800=CARTESIAN_POINT('Ctrl Pts',(17.0209586919664,-20.1958709981426,
-1.20707124330506));
#112801=CARTESIAN_POINT('Ctrl Pts',(17.0245195218161,-20.2007602167504,
-1.20670834888374));
#112802=CARTESIAN_POINT('Ctrl Pts',(17.0319301924233,-20.2108443816476,
-1.20595919785515));
#112803=CARTESIAN_POINT('Ctrl Pts',(17.0357829816325,-20.2160370908435,
-1.2055730610832));
#112804=CARTESIAN_POINT('Ctrl Pts',(17.0448505163654,-20.228141837466,-1.20467201801022));
#112805=CARTESIAN_POINT('Ctrl Pts',(17.0500840206145,-20.2350397285979,
-1.20415785261978));
#112806=CARTESIAN_POINT('Ctrl Pts',(17.0671668213754,-20.2572707208069,
-1.20249829610703));
#112807=CARTESIAN_POINT('Ctrl Pts',(17.0791845743477,-20.2724735680331,
-1.20135956747992));
#112808=CARTESIAN_POINT('Ctrl Pts',(17.1414403955605,-20.3490441937779,
-1.19560092451776));
#112809=CARTESIAN_POINT('Ctrl Pts',(17.1948923638484,-20.4077225769487,
-1.19111361433064));
#112810=CARTESIAN_POINT('Ctrl Pts',(17.3679313979148,-20.5774658583777,
-1.17766507016939));
#112811=CARTESIAN_POINT('Ctrl Pts',(17.4971417822176,-20.6778211704038,
-1.16906404353162));
#112812=CARTESIAN_POINT('Ctrl Pts',(17.6888228912938,-20.7940168254065,
-1.1565347881372));
#112813=CARTESIAN_POINT('Ctrl Pts',(17.742406533583,-20.8234064506605,-1.15304834159926));
#112814=CARTESIAN_POINT('Ctrl Pts',(17.8053530517049,-20.8544686356864,
-1.14888518455534));
#112815=CARTESIAN_POINT('Ctrl Pts',(17.813551860981,-20.8584488666064,-1.14834164637157));
#112816=CARTESIAN_POINT('Ctrl Pts',(17.8258415152737,-20.8643173022009,
-1.14752461591503));
#112817=CARTESIAN_POINT('Ctrl Pts',(17.8299132262763,-20.8662456483934,
-1.14725355039542));
#112818=CARTESIAN_POINT('Ctrl Pts',(17.837219374842,-20.8696773012974,-1.1467664365007));
#112819=CARTESIAN_POINT('Ctrl Pts',(17.8404514818805,-20.8711854436304,
-1.14655069120268));
#112820=CARTESIAN_POINT('Ctrl Pts',(17.8474676197136,-20.8744376970473,
-1.14608179516534));
#112821=CARTESIAN_POINT('Ctrl Pts',(17.8512529429665,-20.8761787840357,
-1.14582846849364));
#112822=CARTESIAN_POINT('Ctrl Pts',(17.861859250324,-20.8810193481851,-1.14511773346867));
#112823=CARTESIAN_POINT('Ctrl Pts',(17.868691506005,-20.8840937708311,-1.1446588325517));
#112824=CARTESIAN_POINT('Ctrl Pts',(17.9088205241138,-20.9018957438009,
-1.14195787695079));
#112825=CARTESIAN_POINT('Ctrl Pts',(17.9424743184824,-20.915797674474,-1.13967023166682));
#112826=CARTESIAN_POINT('Ctrl Pts',(18.0526132122882,-20.9580036619708,
-1.13214925938801));
#112827=CARTESIAN_POINT('Ctrl Pts',(18.1303766047942,-20.9827574167094,
-1.12678910459031));
#112828=CARTESIAN_POINT('Ctrl Pts',(18.3869095222611,-21.0483780084675,
-1.10930507020568));
#112829=CARTESIAN_POINT('Ctrl Pts',(18.5696370504609,-21.0705570508792,
-1.09724050439611));
#112830=CARTESIAN_POINT('Ctrl Pts',(18.7752747831385,-21.0687152294627,
-1.08459112606208));
#112831=CARTESIAN_POINT('Ctrl Pts',(18.7975852188531,-21.0681625528546,
-1.08322945502247));
#112832=CARTESIAN_POINT('Ctrl Pts',(18.8283696560096,-21.066912646581,-1.08136475180797));
#112833=CARTESIAN_POINT('Ctrl Pts',(18.8368538201628,-21.0665170204114,
-1.08085232480144));
#112834=CARTESIAN_POINT('Ctrl Pts',(18.8514156250629,-21.0657501370288,
-1.07997530663869));
#112835=CARTESIAN_POINT('Ctrl Pts',(18.85749441757,-21.0654037003922,-1.07960994175069));
#112836=CARTESIAN_POINT('Ctrl Pts',(18.8700069918549,-21.0646364256818,
-1.07885937747905));
#112837=CARTESIAN_POINT('Ctrl Pts',(18.8764405208141,-21.0642124108148,
-1.07847428179653));
#112838=CARTESIAN_POINT('Ctrl Pts',(18.8913800445021,-21.0631592235079,
-1.07758189314619));
#112839=CARTESIAN_POINT('Ctrl Pts',(18.899884411973,-21.0625080219041,-1.07707529684525));
#112840=CARTESIAN_POINT('Ctrl Pts',(18.9269811211416,-21.060268359596,-1.07546547260716));
#112841=CARTESIAN_POINT('Ctrl Pts',(18.945556820596,-21.0584854459138,-1.07436835009053));
#112842=CARTESIAN_POINT('Ctrl Pts',(19.1238251993047,-21.0389931045081,
-1.06389558349427));
#112843=CARTESIAN_POINT('Ctrl Pts',(19.2810393471936,-21.0034044022969,
-1.05514839338973));
#112844=CARTESIAN_POINT('Ctrl Pts',(19.5595042799313,-20.9060389797379,
-1.03912865068673));
#112845=CARTESIAN_POINT('Ctrl Pts',(19.6817561718178,-20.8497549827405,
-1.03186595151421));
#112846=CARTESIAN_POINT('Ctrl Pts',(19.8113918545858,-20.7744054540267,
-1.02307441290294));
#112847=CARTESIAN_POINT('Ctrl Pts',(19.8248594179145,-20.7663760759782,
-1.02214689119972));
#112848=CARTESIAN_POINT('Ctrl Pts',(19.8431752333489,-20.7551785309911,
-1.02086416263513));
#112849=CARTESIAN_POINT('Ctrl Pts',(19.8481018917498,-20.7521387407391,
-1.02051699370807));
#112850=CARTESIAN_POINT('Ctrl Pts',(19.8559115710803,-20.7472757621879,
-1.01996316072993));
#112851=CARTESIAN_POINT('Ctrl Pts',(19.8588028021005,-20.7454657207846,
-1.01975735781224));
#112852=CARTESIAN_POINT('Ctrl Pts',(19.8647626891617,-20.7417144816413,
-1.01933150799062));
#112853=CARTESIAN_POINT('Ctrl Pts',(19.8678307177431,-20.7397723814043,
-1.01911139811555));
#112854=CARTESIAN_POINT('Ctrl Pts',(19.8751293409624,-20.7351259178681,
-1.01858566864822));
#112855=CARTESIAN_POINT('Ctrl Pts',(19.8793553252695,-20.732414387007,-1.01827957599067));
#112856=CARTESIAN_POINT('Ctrl Pts',(19.8935793752587,-20.7232161673964,
-1.01724370885702));
#112857=CARTESIAN_POINT('Ctrl Pts',(19.9035320866917,-20.7166602285876,
-1.01650952273431));
#112858=CARTESIAN_POINT('Ctrl Pts',(19.9273102998622,-20.700707797263,-1.01473382806373));
#112859=CARTESIAN_POINT('Ctrl Pts',(19.9410807094834,-20.691231024301,-1.0136876734955));
#112860=CARTESIAN_POINT('Ctrl Pts',(19.9923045130314,-20.655077542099,-1.00973306970564));
#112861=CARTESIAN_POINT('Ctrl Pts',(20.0289958667914,-20.6273472837901,
-1.00677231121293));
#112862=CARTESIAN_POINT('Ctrl Pts',(20.1225743842928,-20.5517117391419,
-0.998935572451693));
#112863=CARTESIAN_POINT('Ctrl Pts',(20.1778923894249,-20.5019647368871,
-0.994011769524073));
#112864=CARTESIAN_POINT('Ctrl Pts',(20.3402766587832,-20.3396818760092,
-0.978844830573222));
#112865=CARTESIAN_POINT('Ctrl Pts',(20.4376925866136,-20.2181887035235,
-0.968729192508623));
#112866=CARTESIAN_POINT('Ctrl Pts',(20.5337902831701,-20.0669067254841,
-0.957687395765254));
#112867=CARTESIAN_POINT('Ctrl Pts',(20.5462827863953,-20.0464830953269,
-0.956225129294907));
#112868=CARTESIAN_POINT('Ctrl Pts',(20.563346207969,-20.017493084651,-0.954188288628662));
#112869=CARTESIAN_POINT('Ctrl Pts',(20.5682083837791,-20.0091010698254,
-0.953603141143982));
#112870=CARTESIAN_POINT('Ctrl Pts',(20.5759803176351,-19.9954718001044,
-0.952659943306616));
#112871=CARTESIAN_POINT('Ctrl Pts',(20.5789257745204,-19.9902551593064,
-0.952300605547992));
#112872=CARTESIAN_POINT('Ctrl Pts',(20.5850180255667,-19.979357505265,-0.951553392589612));
#112873=CARTESIAN_POINT('Ctrl Pts',(20.5881609056978,-19.9736743668263,
-0.951165660915609));
#112874=CARTESIAN_POINT('Ctrl Pts',(20.5955277531521,-19.9602072475418,
-0.950251395307535));
#112875=CARTESIAN_POINT('Ctrl Pts',(20.5997291470569,-19.9524110071407,
-0.949725671690242));
#112876=CARTESIAN_POINT('Ctrl Pts',(20.6135042252298,-19.9264609146362,
-0.947987337117727));
#112877=CARTESIAN_POINT('Ctrl Pts',(20.6228630273264,-19.908193868702,-0.946782330914329));
#112878=CARTESIAN_POINT('Ctrl Pts',(20.6710793542249,-19.8106111351768,
-0.940438850966872));
#112879=CARTESIAN_POINT('Ctrl Pts',(20.7052127833459,-19.7290535594662,
-0.935466841537171));
#112880=CARTESIAN_POINT('Ctrl Pts',(20.7770356124094,-19.5219342745485,
-0.923366577005673));
#112881=CARTESIAN_POINT('Ctrl Pts',(20.8083554811537,-19.3945691508358,
-0.916389496580278));
#112882=CARTESIAN_POINT('Ctrl Pts',(20.8332930141252,-19.2278269740611,
-0.907089596115496));
#112883=CARTESIAN_POINT('Ctrl Pts',(20.8378738659814,-19.1903824739513,
-0.904989166941394));
#112884=CARTESIAN_POINT('Ctrl Pts',(20.845804004131,-19.1071688939514,-0.900257380576004));
#112885=CARTESIAN_POINT('Ctrl Pts',(20.8486701922348,-19.0613747650289,
-0.897610771994247));
#112886=CARTESIAN_POINT('Ctrl Pts',(20.8502754956742,-19.0079035291881,
-0.894433888747696));
#112887=CARTESIAN_POINT('Ctrl Pts',(20.850463173625,-19.0002784515828,-0.893978808073013));
#112888=CARTESIAN_POINT('Ctrl Pts',(20.8506981094217,-18.9880463513708,
-0.893245242277728));
#112889=CARTESIAN_POINT('Ctrl Pts',(20.8507715424004,-18.9834398193474,
-0.89296818350772));
#112890=CARTESIAN_POINT('Ctrl Pts',(20.8508753307636,-18.9752520947348,
-0.892474250722606));
#112891=CARTESIAN_POINT('Ctrl Pts',(20.8509116364345,-18.9716710254737,
-0.892257712695064));
#112892=CARTESIAN_POINT('Ctrl Pts',(20.8509695804583,-18.9640473296703,
-0.891795630695948));
#112893=CARTESIAN_POINT('Ctrl Pts',(20.8509887258639,-18.9600047904858,
-0.891549955828478));
#112894=CARTESIAN_POINT('Ctrl Pts',(20.8510092763643,-18.9490248631197,
-0.890880955692545));
#112895=CARTESIAN_POINT('Ctrl Pts',(20.8509881596246,-18.942087554154,-0.890456401136245));
#112896=CARTESIAN_POINT('Ctrl Pts',(20.8507068074548,-18.9067389251845,
-0.88828401798507));
#112897=CARTESIAN_POINT('Ctrl Pts',(20.849908728059,-18.8783362744689,-0.886508599459404));
#112898=CARTESIAN_POINT('Ctrl Pts',(20.8458846388466,-18.7949465021971,
-0.881224624397769));
#112899=CARTESIAN_POINT('Ctrl Pts',(20.8410841553577,-18.7400611889243,
-0.877655877078888));
#112900=CARTESIAN_POINT('Ctrl Pts',(20.8165299602159,-18.546613284839,-0.864885057049364));
#112901=CARTESIAN_POINT('Ctrl Pts',(20.7851879933606,-18.4098725167902,
-0.855533051259325));
#112902=CARTESIAN_POINT('Ctrl Pts',(20.7117633298357,-18.1915296121857,
-0.840658554401902));
#112903=CARTESIAN_POINT('Ctrl Pts',(20.6774831622946,-18.1077607332038,
-0.834959698999613));
#112904=CARTESIAN_POINT('Ctrl Pts',(20.6319419398103,-18.0140799685371,
-0.828603961796962));
#112905=CARTESIAN_POINT('Ctrl Pts',(20.6258176663965,-18.0017876430153,
-0.827770211360294));
#112906=CARTESIAN_POINT('Ctrl Pts',(20.6158033006481,-17.9821679874033,
-0.826439617841622));
#112907=CARTESIAN_POINT('Ctrl Pts',(20.6119890786087,-17.9748025692469,
-0.825940132343313));
#112908=CARTESIAN_POINT('Ctrl Pts',(20.605139317047,-17.9617636368225,-0.82505589389912));
#112909=CARTESIAN_POINT('Ctrl Pts',(20.6021210313848,-17.9560812220505,
-0.824670538119259));
#112910=CARTESIAN_POINT('Ctrl Pts',(20.5957777920921,-17.9442693433204,
-0.82386946804403));
#112911=CARTESIAN_POINT('Ctrl Pts',(20.5924483619717,-17.9381423614674,
-0.823453918618515));
#112912=CARTESIAN_POINT('Ctrl Pts',(20.5837221242851,-17.9222713311964,
-0.822377370762704));
#112913=CARTESIAN_POINT('Ctrl Pts',(20.578278534909,-17.9125531464928,-0.821718050165515));
#112914=CARTESIAN_POINT('Ctrl Pts',(20.5542933230677,-17.870515118424,-0.818864946127468));
#112915=CARTESIAN_POINT('Ctrl Pts',(20.5349762835991,-17.8386438096503,
-0.8166992301243));
#112916=CARTESIAN_POINT('Ctrl Pts',(20.481403120302,-17.7552994113448,-0.811013082640622));
#112917=CARTESIAN_POINT('Ctrl Pts',(20.4457162163399,-17.7047877418501,
-0.807543794594892));
#112918=CARTESIAN_POINT('Ctrl Pts',(20.3211978524967,-17.5439757539065,
-0.796291211123318));
#112919=CARTESIAN_POINT('Ctrl Pts',(20.2235242093855,-17.4410252810488,
-0.788766688059283));
#112920=CARTESIAN_POINT('Ctrl Pts',(20.0589236171188,-17.2991214866803,
-0.77673606087605));
#112921=CARTESIAN_POINT('Ctrl Pts',(19.998927949183,-17.2527693896341,-0.772455130894074));
#112922=CARTESIAN_POINT('Ctrl Pts',(19.9287599195456,-17.204336377034,-0.767402196982563));
#112923=CARTESIAN_POINT('Ctrl Pts',(19.9208987289038,-17.1989880764515,
-0.766835464318208));
#112924=CARTESIAN_POINT('Ctrl Pts',(19.9091922916748,-17.1911385300126,
-0.765990160622017));
#112925=CARTESIAN_POINT('Ctrl Pts',(19.905374388484,-17.1885964500448,-0.765714263548012));
#112926=CARTESIAN_POINT('Ctrl Pts',(19.8985613166124,-17.1840919814935,
-0.765221489398647));
#112927=CARTESIAN_POINT('Ctrl Pts',(19.8955694031899,-17.1821247661727,
-0.765004940084503));
#112928=CARTESIAN_POINT('Ctrl Pts',(19.8891167829349,-17.1779055082966,
-0.764537575181715));
#112929=CARTESIAN_POINT('Ctrl Pts',(19.885654518553,-17.1756560251639,-0.764286600560479));
#112930=CARTESIAN_POINT('Ctrl Pts',(19.8760707030928,-17.1694690783995,
-0.763591375973212));
#112931=CARTESIAN_POINT('Ctrl Pts',(19.869935459412,-17.1655530777967,-0.76314574640617));
#112932=CARTESIAN_POINT('Ctrl Pts',(19.8360557010601,-17.1441734118384,
-0.76068232189865));
#112933=CARTESIAN_POINT('Ctrl Pts',(19.8079302154371,-17.1273254097837,
-0.758627825383906));
#112934=CARTESIAN_POINT('Ctrl Pts',(19.637111887861,-17.0303175488475,-0.746145431491577));
#112935=CARTESIAN_POINT('Ctrl Pts',(19.4859089384337,-16.9662739910768,
-0.735128286201479));
#112936=CARTESIAN_POINT('Ctrl Pts',(19.2190442627122,-16.8881421578079,
-0.716988267455996));
#112937=CARTESIAN_POINT('Ctrl Pts',(19.1068116667028,-16.8649456380465,
-0.709708815586819));
#112938=CARTESIAN_POINT('Ctrl Pts',(18.9790782211547,-16.8491854089419,
-0.701850773645383));
#112939=CARTESIAN_POINT('Ctrl Pts',(18.9649013265773,-16.8475815216944,
-0.700984207421549));
#112940=CARTESIAN_POINT('Ctrl Pts',(18.9422949865791,-16.8452551781684,
-0.699611052341453));
#112941=CARTESIAN_POINT('Ctrl Pts',(18.9338757416618,-16.8444397430016,
-0.699101558925369));
#112942=CARTESIAN_POINT('Ctrl Pts',(18.9190082003776,-16.8430896587684,
-0.69820514700346));
#112943=CARTESIAN_POINT('Ctrl Pts',(18.9125619584257,-16.8425340746999,
-0.69781757632356));
#112944=CARTESIAN_POINT('Ctrl Pts',(18.8992136717395,-16.8414452475454,
-0.69701725563942));
#112945=CARTESIAN_POINT('Ctrl Pts',(18.8923113478295,-16.8409162879381,
-0.6966046444111));
#112946=CARTESIAN_POINT('Ctrl Pts',(18.8745658966637,-16.8396438862354,
-0.695546941577965));
#112947=CARTESIAN_POINT('Ctrl Pts',(18.8637193293942,-16.8389500656871,
-0.694903409364044));
#112948=CARTESIAN_POINT('Ctrl Pts',(18.8182406794367,-16.8363924433478,
-0.692217110239066));
#112949=CARTESIAN_POINT('Ctrl Pts',(18.7835696528897,-16.8352962233687,
-0.69019837930424));
#112950=CARTESIAN_POINT('Ctrl Pts',(18.693002206864,-16.8346593773351,-0.684989112666923));
#112951=CARTESIAN_POINT('Ctrl Pts',(18.6371224131308,-16.8364793706412,
-0.681839177258327));
#112952=CARTESIAN_POINT('Ctrl Pts',(18.3834474860446,-16.8548155386015,
-0.667705158163168));
#112953=CARTESIAN_POINT('Ctrl Pts',(18.1885440452532,-16.896877579339,-0.657394732512601));
#112954=CARTESIAN_POINT('Ctrl Pts',(17.9724290817017,-16.9764704756795,
-0.644170672438002));
#112955=CARTESIAN_POINT('Ctrl Pts',(17.9427414385785,-16.9881729180789,
-0.642310099739248));
#112956=CARTESIAN_POINT('Ctrl Pts',(17.9070460604945,-17.0031842892043,
-0.640006155137102));
#112957=CARTESIAN_POINT('Ctrl Pts',(17.90077359204,-17.0058578564428,-0.63959876083637));
#112958=CARTESIAN_POINT('Ctrl Pts',(17.8904623225333,-17.0103119024413,
-0.638924681610809));
#112959=CARTESIAN_POINT('Ctrl Pts',(17.8864159253901,-17.0120748166069,
-0.638659043197406));
#112960=CARTESIAN_POINT('Ctrl Pts',(17.879124972349,-17.0152784686418,-0.638178343238376));
#112961=CARTESIAN_POINT('Ctrl Pts',(17.8758784976345,-17.0167147264671,
-0.637963557868887));
#112962=CARTESIAN_POINT('Ctrl Pts',(17.8695669221827,-17.0195260056022,
-0.63754452175214));
#112963=CARTESIAN_POINT('Ctrl Pts',(17.866501524906,-17.0209001371259,-0.637340333511754));
#112964=CARTESIAN_POINT('Ctrl Pts',(17.8574579487995,-17.0249799969133,
-0.636735978479423));
#112965=CARTESIAN_POINT('Ctrl Pts',(17.8514891312339,-17.0277062013054,
-0.636334570302513));
#112966=CARTESIAN_POINT('Ctrl Pts',(17.8231334872806,-17.0408170654135,
-0.63441590105685));
#112967=CARTESIAN_POINT('Ctrl Pts',(17.8009177279784,-17.0515644280766,
-0.632877779752791));
#112968=CARTESIAN_POINT('Ctrl Pts',(17.738720024919,-17.0830073851841,-0.628482638598404));
#112969=CARTESIAN_POINT('Ctrl Pts',(17.699204538176,-17.1045927760092,-0.625584859587855));
#112970=CARTESIAN_POINT('Ctrl Pts',(17.5784806017701,-17.1756272124288,
-0.616463122397769));
#112971=CARTESIAN_POINT('Ctrl Pts',(17.4998931148633,-17.2292971844216,
-0.610137970553651));
#112972=CARTESIAN_POINT('Ctrl Pts',(17.307368059534,-17.3807338437067,-0.593981628709136));
#112973=CARTESIAN_POINT('Ctrl Pts',(17.199711591409,-17.4856674460666,-0.584307127741038));
#112974=CARTESIAN_POINT('Ctrl Pts',(17.0950142926375,-17.6119945888665,
-0.574290992265421));
#112975=CARTESIAN_POINT('Ctrl Pts',(17.086106874914,-17.6229639153124,-0.573432878400448));
#112976=CARTESIAN_POINT('Ctrl Pts',(17.072093705984,-17.6405783798368,-0.572073056529783));
#112977=CARTESIAN_POINT('Ctrl Pts',(17.0669165480973,-17.6471659249212,
-0.571568472289585));
#112978=CARTESIAN_POINT('Ctrl Pts',(17.0578486721638,-17.6588461827973,
-0.570680710981957));
#112979=CARTESIAN_POINT('Ctrl Pts',(17.0539417418264,-17.6639261204009,
-0.570296888066272));
#112980=CARTESIAN_POINT('Ctrl Pts',(17.0459029806981,-17.6744772186052,
-0.569504345809204));
#112981=CARTESIAN_POINT('Ctrl Pts',(17.0417745351756,-17.6799508730127,
-0.569095763517996));
#112982=CARTESIAN_POINT('Ctrl Pts',(17.0312343077408,-17.6940676455551,
-0.568048528131414));
#112983=CARTESIAN_POINT('Ctrl Pts',(17.0248616579755,-17.7027398407741,
-0.56741141622733));
#112984=CARTESIAN_POINT('Ctrl Pts',(16.9984537680377,-17.739257234796,-0.564754091848449));
#112985=CARTESIAN_POINT('Ctrl Pts',(16.979030031329,-17.7675396399212,-0.562757572942994));
#112986=CARTESIAN_POINT('Ctrl Pts',(16.9301570456348,-17.8425458372623,
-0.55760883954137));
#112987=CARTESIAN_POINT('Ctrl Pts',(16.9018328811112,-17.8899725785667,
-0.554496496736844));
#112988=CARTESIAN_POINT('Ctrl Pts',(16.8405517958169,-18.0023478892813,
-0.547383536926009));
#112989=CARTESIAN_POINT('Ctrl Pts',(16.8090263232568,-18.067996473509,-0.543420742657022));
#112990=CARTESIAN_POINT('Ctrl Pts',(16.7673556016827,-18.1676283178345,
-0.537557188721337));
#112991=CARTESIAN_POINT('Ctrl Pts',(16.7545802832847,-18.2004504712821,
-0.535648363153797));
#112992=CARTESIAN_POINT('Ctrl Pts',(16.7287365521522,-18.2720856476005,
-0.531505691853217));
#112993=CARTESIAN_POINT('Ctrl Pts',(16.7159637403136,-18.3109894545521,
-0.529270380739138));
#112994=CARTESIAN_POINT('Ctrl Pts',(16.6989488456493,-18.3683787119344,
-0.525964161640086));
#112995=CARTESIAN_POINT('Ctrl Pts',(16.6938140192241,-18.3865902848655,
-0.524913687915817));
#112996=CARTESIAN_POINT('Ctrl Pts',(16.6732969948426,-18.4632790246769,
-0.520475810133252));
#112997=CARTESIAN_POINT('Ctrl Pts',(16.6601810645928,-18.5223272734326,
-0.517024246174424));
#112998=CARTESIAN_POINT('Ctrl Pts',(16.6480273156646,-18.5907673934646,
-0.512901039303712));
#112999=CARTESIAN_POINT('Ctrl Pts',(16.6465009452968,-18.5996951238406,
-0.51236080294181));
#113000=CARTESIAN_POINT('Ctrl Pts',(16.644305601677,-18.6130510721475,-0.511548680017965));
#113001=CARTESIAN_POINT('Ctrl Pts',(16.6435932922695,-18.6174721992162,
-0.511279207093751));
#113002=CARTESIAN_POINT('Ctrl Pts',(16.6423403650114,-18.625409087299,-0.510794240062401));
#113003=CARTESIAN_POINT('Ctrl Pts',(16.6417945762315,-18.6289239762063,
-0.510579043265837));
#113004=CARTESIAN_POINT('Ctrl Pts',(16.6407479422931,-18.6357782032962,
-0.510158565565197));
#113005=CARTESIAN_POINT('Ctrl Pts',(16.6402462293206,-18.6391173555435,
-0.509953340961359));
#113006=CARTESIAN_POINT('Ctrl Pts',(16.6391504857787,-18.6465307459401,
-0.509496887874436));
#113007=CARTESIAN_POINT('Ctrl Pts',(16.6385603498353,-18.6506055337683,
-0.50924544453661));
#113008=CARTESIAN_POINT('Ctrl Pts',(16.6371204756496,-18.6607562875997,
-0.508617738797099));
#113009=CARTESIAN_POINT('Ctrl Pts',(16.6362852620975,-18.6668342307324,
-0.508240701530483));
#113010=CARTESIAN_POINT('Ctrl Pts',(16.6323977830372,-18.6960654138083,
-0.5064219570469));
#113011=CARTESIAN_POINT('Ctrl Pts',(16.6297024906904,-18.7192634938548,
-0.504962249722664));
#113012=CARTESIAN_POINT('Ctrl Pts',(16.6205187004321,-18.8116103989568,
-0.499098991253069));
#113013=CARTESIAN_POINT('Ctrl Pts',(16.6170514726509,-18.881010439068,-0.494577327914004));
#113014=CARTESIAN_POINT('Ctrl Pts',(16.6170005688548,-18.9504480557866,
-0.49001046713057));
#113015=CARTESIAN_POINT('Ctrl Pts',(16.6170006157907,-18.95038529957,-0.489056278967188));
#113016=CARTESIAN_POINT('Ctrl Pts',(16.6169459705064,-19.0220295693798,
-0.484732818390677));
#113017=CARTESIAN_POINT('Ctrl Pts',(16.620532458768,-19.0938083580375,-0.480409357814167));
#113018=CARTESIAN_POINT('Ctrl Pts',(16.6277745422071,-19.1653150743503,
-0.476085897237656));
#113019=CARTESIAN_POINT('Ctrl Pts',(16.6350090271023,-19.2367467643357,
-0.471766972925506));
#113020=CARTESIAN_POINT('Ctrl Pts',(16.6458914554201,-19.3079064569402,
-0.467448048613356));
#113021=CARTESIAN_POINT('Ctrl Pts',(16.6603842666415,-19.3783880748427,
-0.463129124301205));
#113022=CARTESIAN_POINT('Ctrl Pts',(16.6748666504828,-19.4488189821819,
-0.458813307396227));
#113023=CARTESIAN_POINT('Ctrl Pts',(16.6929541651561,-19.5185722974559,
-0.454497490491248));
#113024=CARTESIAN_POINT('Ctrl Pts',(16.7145577237479,-19.5872494729519,
-0.45018167358627));
#113025=CARTESIAN_POINT('Ctrl Pts',(16.7241553569732,-19.6177601102879,
-0.448264321519214));
#113026=CARTESIAN_POINT('Ctrl Pts',(16.7344462702044,-19.6480584841912,
-0.446346969452159));
#113027=CARTESIAN_POINT('Ctrl Pts',(16.7454194499637,-19.6781104571739,
-0.444429617385103));
#113028=CARTESIAN_POINT('Origin',(-18.734,-18.952,0.));
#113029=CARTESIAN_POINT('',(-20.8509997094775,-18.9508909138291,-0.710943720977502));
#113030=CARTESIAN_POINT('Ctrl Pts',(-20.7225805821191,-19.6781103693095,
-0.666446455478431));
#113031=CARTESIAN_POINT('Ctrl Pts',(-20.7478889918429,-19.6087988510222,
-0.670880806094382));
#113032=CARTESIAN_POINT('Ctrl Pts',(-20.7695971667487,-19.5380870993955,
-0.675315156710334));
#113033=CARTESIAN_POINT('Ctrl Pts',(-20.7875590822766,-19.4663773863607,
-0.679749507326285));
#113034=CARTESIAN_POINT('Ctrl Pts',(-20.8055066130117,-19.3947251020211,
-0.684180306694308));
#113035=CARTESIAN_POINT('Ctrl Pts',(-20.8197137318595,-19.3220768932863,
-0.68861110606233));
#113036=CARTESIAN_POINT('Ctrl Pts',(-20.8300841804326,-19.2488503133574,
-0.693041905430352));
#113037=CARTESIAN_POINT('Ctrl Pts',(-20.8404495313235,-19.175659728576,
-0.697470526801298));
#113038=CARTESIAN_POINT('Ctrl Pts',(-20.8469818946778,-19.1018917970174,
-0.701899148172244));
#113039=CARTESIAN_POINT('Ctrl Pts',(-20.8496363361419,-19.0279729767482,
-0.70632776954319));
#113040=CARTESIAN_POINT('Ctrl Pts',(-20.8505585774639,-19.0022911180789,
-0.707866420021294));
#113041=CARTESIAN_POINT('Ctrl Pts',(-20.8510131736829,-18.9765910979418,
-0.709405070499398));
#113042=CARTESIAN_POINT('Ctrl Pts',(-20.8509997094775,-18.9508909138291,
-0.710943720977502));
#113043=CARTESIAN_POINT('Ctrl Pts',(-20.8509997572023,-18.9509860940746,
-0.712619188017889));
#113044=CARTESIAN_POINT('Ctrl Pts',(-20.850964631018,-18.8776438618634,
-0.716785661483279));
#113045=CARTESIAN_POINT('Ctrl Pts',(-20.8471182042979,-18.8043479163262,
-0.720847520086871));
#113046=CARTESIAN_POINT('Ctrl Pts',(-20.8225250941853,-18.5696299416392,
-0.733763884425625));
#113047=CARTESIAN_POINT('Ctrl Pts',(-20.7869923924286,-18.4103781101525,
-0.742358139260776));
#113048=CARTESIAN_POINT('Ctrl Pts',(-20.7229676898254,-18.2262294227371,
-0.753553850662875));
#113049=CARTESIAN_POINT('Ctrl Pts',(-20.7116463931708,-18.1959246812705,
-0.755440714754925));
#113050=CARTESIAN_POINT('Ctrl Pts',(-20.6969536994598,-18.1591860537959,
-0.757796644379626));
#113051=CARTESIAN_POINT('Ctrl Pts',(-20.6942371115394,-18.1524928751802,
-0.758228674046915));
#113052=CARTESIAN_POINT('Ctrl Pts',(-20.6899236894109,-18.1420195311309,
-0.758909328814416));
#113053=CARTESIAN_POINT('Ctrl Pts',(-20.6883499983137,-18.1382298099701,
-0.75915657360869));
#113054=CARTESIAN_POINT('Ctrl Pts',(-20.6853861958599,-18.1311506425931,
-0.75962025348826));
#113055=CARTESIAN_POINT('Ctrl Pts',(-20.6839987756849,-18.1278601289272,
-0.759836524939919));
#113056=CARTESIAN_POINT('Ctrl Pts',(-20.6808111784495,-18.1203532880343,
-0.760331610884589));
#113057=CARTESIAN_POINT('Ctrl Pts',(-20.6790056308094,-18.1161392979295,
-0.760610749093168));
#113058=CARTESIAN_POINT('Ctrl Pts',(-20.6734109853909,-18.1031981677212,
-0.761471662144984));
#113059=CARTESIAN_POINT('Ctrl Pts',(-20.6695767924482,-18.0944908201619,
-0.762056084851175));
#113060=CARTESIAN_POINT('Ctrl Pts',(-20.6165813810053,-17.9763061593527,
-0.77005598901314));
#113061=CARTESIAN_POINT('Ctrl Pts',(-20.5582617224411,-17.871188441333,
-0.777951515509893));
#113062=CARTESIAN_POINT('Ctrl Pts',(-20.4306702152987,-17.6812337367286,
-0.793068874262596));
#113063=CARTESIAN_POINT('Ctrl Pts',(-20.363095503531,-17.5956858642857,
-0.800262887893773));
#113064=CARTESIAN_POINT('Ctrl Pts',(-20.252283159863,-17.4756965346801,
-0.810755849071076));
#113065=CARTESIAN_POINT('Ctrl Pts',(-20.2137969225058,-17.4371212794387,
-0.814203379954689));
#113066=CARTESIAN_POINT('Ctrl Pts',(-20.1572924335114,-17.3846970365266,
-0.818993217678231));
#113067=CARTESIAN_POINT('Ctrl Pts',(-20.1404764348063,-17.3695891713637,
-0.820386945875824));
#113068=CARTESIAN_POINT('Ctrl Pts',(-20.114318725804,-17.3468349724094,
-0.822507372087951));
#113069=CARTESIAN_POINT('Ctrl Pts',(-20.1051486143512,-17.3389947187231,
-0.823242027532029));
#113070=CARTESIAN_POINT('Ctrl Pts',(-20.0880140846261,-17.3245967695061,
-0.824598863731232));
#113071=CARTESIAN_POINT('Ctrl Pts',(-20.0800678308926,-17.3180181101005,
-0.825221892191775));
#113072=CARTESIAN_POINT('Ctrl Pts',(-20.0669001276875,-17.307277889046,
-0.826244239948318));
#113073=CARTESIAN_POINT('Ctrl Pts',(-20.0617065809242,-17.3030825341428,
-0.826644924850156));
#113074=CARTESIAN_POINT('Ctrl Pts',(-20.0514495199719,-17.2948767448298,
-0.827431313417878));
#113075=CARTESIAN_POINT('Ctrl Pts',(-20.0463873291951,-17.2908647797079,
-0.827817076068002));
#113076=CARTESIAN_POINT('Ctrl Pts',(-20.0346550516866,-17.281653642031,
-0.828705779615124));
#113077=CARTESIAN_POINT('Ctrl Pts',(-20.0279719855212,-17.2764711214339,
-0.82920805457678));
#113078=CARTESIAN_POINT('Ctrl Pts',(-20.0099118661412,-17.2626385338318,
-0.830554923825369));
#113079=CARTESIAN_POINT('Ctrl Pts',(-19.9984778539664,-17.2540633035146,
-0.831396577707444));
#113080=CARTESIAN_POINT('Ctrl Pts',(-19.8930995769677,-17.1766870392063,
-0.839055562750339));
#113081=CARTESIAN_POINT('Ctrl Pts',(-19.7937099858338,-17.1156264259946,
-0.845558675082553));
#113082=CARTESIAN_POINT('Ctrl Pts',(-19.5445352122423,-16.9895467831458,
-0.860849606959898));
#113083=CARTESIAN_POINT('Ctrl Pts',(-19.39130540912,-16.933057766199,-0.869452606281301));
#113084=CARTESIAN_POINT('Ctrl Pts',(-19.2014072603363,-16.8869853199322,
-0.880671120996706));
#113085=CARTESIAN_POINT('Ctrl Pts',(-19.1695035487123,-16.8800223045043,
-0.882575372180294));
#113086=CARTESIAN_POINT('Ctrl Pts',(-19.1303340925041,-16.8724180984619,
-0.884951048685638));
#113087=CARTESIAN_POINT('Ctrl Pts',(-19.1232076227952,-16.8710725574915,
-0.885384795887963));
#113088=CARTESIAN_POINT('Ctrl Pts',(-19.1120279494661,-16.8690211726241,
-0.886067813576971));
#113089=CARTESIAN_POINT('Ctrl Pts',(-19.1079792850815,-16.8682904666097,
-0.886315693419612));
#113090=CARTESIAN_POINT('Ctrl Pts',(-19.1004106025692,-16.8669472342115,
-0.88678011651294));
#113091=CARTESIAN_POINT('Ctrl Pts',(-19.0968911554678,-16.8663318158353,
-0.886996493281382));
#113092=CARTESIAN_POINT('Ctrl Pts',(-19.0888568438837,-16.8649478696211,
-0.887491394053295));
#113093=CARTESIAN_POINT('Ctrl Pts',(-19.0843410509844,-16.8641850844352,
-0.887770238752649));
#113094=CARTESIAN_POINT('Ctrl Pts',(-19.0704611381452,-16.8618868577665,
-0.888629316287147));
#113095=CARTESIAN_POINT('Ctrl Pts',(-19.0610892909,-16.8603997435232,-0.889212180646249));
#113096=CARTESIAN_POINT('Ctrl Pts',(-18.9323061362925,-16.8408512679557,
-0.897257144669816));
#113097=CARTESIAN_POINT('Ctrl Pts',(-18.8115857524508,-16.8329794704031,
-0.905205339547631));
#113098=CARTESIAN_POINT('Ctrl Pts',(-18.5117666877223,-16.8390891261654,
-0.925017373247488));
#113099=CARTESIAN_POINT('Ctrl Pts',(-18.3338128414782,-16.8654584894827,
-0.936778359655229));
#113100=CARTESIAN_POINT('Ctrl Pts',(-18.1406018114183,-16.919752677353,
-0.949107327055617));
#113101=CARTESIAN_POINT('Ctrl Pts',(-18.1200073978207,-16.9258796362289,
-0.950416984134922));
#113102=CARTESIAN_POINT('Ctrl Pts',(-18.0908984537672,-16.9350243273827,
-0.952262298924337));
#113103=CARTESIAN_POINT('Ctrl Pts',(-18.0823049836019,-16.9377845020349,
-0.952806346304224));
#113104=CARTESIAN_POINT('Ctrl Pts',(-18.067525618235,-16.9426360380585,
-0.953740848063025));
#113105=CARTESIAN_POINT('Ctrl Pts',(-18.0613313149609,-16.9447011994352,
-0.95413215877235));
#113106=CARTESIAN_POINT('Ctrl Pts',(-18.0494997399287,-16.9487067274606,
-0.954878945147));
#113107=CARTESIAN_POINT('Ctrl Pts',(-18.0438609256574,-16.9506423105741,
-0.955234574450041));
#113108=CARTESIAN_POINT('Ctrl Pts',(-18.0292418495597,-16.9557295960538,
-0.956155880435101));
#113109=CARTESIAN_POINT('Ctrl Pts',(-18.0202744665804,-16.9589181041099,
-0.9567203321157));
#113110=CARTESIAN_POINT('Ctrl Pts',(-17.9898855188329,-16.9699548183433,
-0.958631094151841));
#113111=CARTESIAN_POINT('Ctrl Pts',(-17.9685689674468,-16.978088943957,
-0.95996788295131));
#113112=CARTESIAN_POINT('Ctrl Pts',(-17.7822653249788,-17.0526520215882,
-0.971630642283501));
#113113=CARTESIAN_POINT('Ctrl Pts',(-17.6261311732976,-17.1392797013109,
-0.981181748730143));
#113114=CARTESIAN_POINT('Ctrl Pts',(-17.413782395421,-17.2948923701231,
-0.995511430765395));
#113115=CARTESIAN_POINT('Ctrl Pts',(-17.3480296005977,-17.3494819905999,
-1.0001909121203));
#113116=CARTESIAN_POINT('Ctrl Pts',(-17.2584705224172,-17.4334805280647,
-1.00720431964912));
#113117=CARTESIAN_POINT('Ctrl Pts',(-17.2318680831641,-17.4597909184569,
-1.00937813157564));
#113118=CARTESIAN_POINT('Ctrl Pts',(-17.2007546230231,-17.4922381763028,
-1.01205292551249));
#113119=CARTESIAN_POINT('Ctrl Pts',(-17.1955599921347,-17.4977138155592,
-1.01250411152458));
#113120=CARTESIAN_POINT('Ctrl Pts',(-17.1875363651409,-17.5062625852512,
-1.01320843434943));
#113121=CARTESIAN_POINT('Ctrl Pts',(-17.184686936081,-17.5093165712382,
-1.01346003182036));
#113122=CARTESIAN_POINT('Ctrl Pts',(-17.179423070408,-17.5149919029403,
-1.01392759838447));
#113123=CARTESIAN_POINT('Ctrl Pts',(-17.1770062080904,-17.5176109201461,
-1.01414337740842));
#113124=CARTESIAN_POINT('Ctrl Pts',(-17.1715619136192,-17.5235405670129,
-1.01463193342264));
#113125=CARTESIAN_POINT('Ctrl Pts',(-17.168538402035,-17.5268547056869,
-1.0149049996497));
#113126=CARTESIAN_POINT('Ctrl Pts',(-17.1596586959676,-17.5366503035713,
-1.01571205547905));
#113127=CARTESIAN_POINT('Ctrl Pts',(-17.1538321408568,-17.543158335492,
-1.01624819093665));
#113128=CARTESIAN_POINT('Ctrl Pts',(-17.1124198293643,-17.5899943291057,
-1.02010494607336));
#113129=CARTESIAN_POINT('Ctrl Pts',(-17.0783450568244,-17.6316260577086,
-1.02352424029672));
#113130=CARTESIAN_POINT('Ctrl Pts',(-16.9526015051071,-17.79778590453,-1.03699530452035));
#113131=CARTESIAN_POINT('Ctrl Pts',(-16.8730915694235,-17.9309151274526,
-1.04738335034069));
#113132=CARTESIAN_POINT('Ctrl Pts',(-16.770102185504,-18.1561071343316,
-1.06345670520847));
#113133=CARTESIAN_POINT('Ctrl Pts',(-16.7370305857035,-18.2431578468464,
-1.06935955476122));
#113134=CARTESIAN_POINT('Ctrl Pts',(-16.7036093562023,-18.3522931717415,
-1.07636851192662));
#113135=CARTESIAN_POINT('Ctrl Pts',(-16.6977313051731,-18.3725655348653,
-1.07765472999939));
#113136=CARTESIAN_POINT('Ctrl Pts',(-16.6897908267291,-18.4015654913221,
-1.079472958303));
#113137=CARTESIAN_POINT('Ctrl Pts',(-16.68747929468,-18.4102230172991,-1.08001302979415));
#113138=CARTESIAN_POINT('Ctrl Pts',(-16.6835816992291,-18.4252018784276,
-1.0809427958372));
#113139=CARTESIAN_POINT('Ctrl Pts',(-16.6819697422263,-18.431516290664,
-1.0813333245803));
#113140=CARTESIAN_POINT('Ctrl Pts',(-16.6789360176397,-18.4436332841626,
-1.0820800471102));
#113141=CARTESIAN_POINT('Ctrl Pts',(-16.6775096067372,-18.449434628222,
-1.08243638763739));
#113142=CARTESIAN_POINT('Ctrl Pts',(-16.6738576842075,-18.4645632476118,
-1.08336263296591));
#113143=CARTESIAN_POINT('Ctrl Pts',(-16.6716709374437,-18.4738998104669,
-1.08393128542887));
#113144=CARTESIAN_POINT('Ctrl Pts',(-16.6643984342844,-18.505929184234,
-1.08587214324255));
#113145=CARTESIAN_POINT('Ctrl Pts',(-16.659623081995,-18.528691272768,-1.08723440551242));
#113146=CARTESIAN_POINT('Ctrl Pts',(-16.622759356728,-18.7200441334948,
-1.09855503281612));
#113147=CARTESIAN_POINT('Ctrl Pts',(-16.6109048184111,-18.8918811289625,
-1.1078004019157));
#113148=CARTESIAN_POINT('Ctrl Pts',(-16.6246444007161,-19.1529064185535,
-1.12201427758092));
#113149=CARTESIAN_POINT('Ctrl Pts',(-16.6350568150434,-19.2421368322252,
-1.12691916895212));
#113150=CARTESIAN_POINT('Ctrl Pts',(-16.6579819809965,-19.3683185976219,
-1.13423619678522));
#113151=CARTESIAN_POINT('Ctrl Pts',(-16.6658979423526,-19.4060104066427,
-1.13647194471781));
#113152=CARTESIAN_POINT('Ctrl Pts',(-16.6766033184645,-19.4508645143586,
-1.1392153657923));
#113153=CARTESIAN_POINT('Ctrl Pts',(-16.678409801845,-19.4582566959017,
-1.13967021507414));
#113154=CARTESIAN_POINT('Ctrl Pts',(-16.6812727194323,-19.4697038432969,
-1.14037902080438));
#113155=CARTESIAN_POINT('Ctrl Pts',(-16.6823014258713,-19.4737657692599,
-1.14063140598727));
#113156=CARTESIAN_POINT('Ctrl Pts',(-16.6842271484725,-19.4812758749446,
-1.14109970022834));
#113157=CARTESIAN_POINT('Ctrl Pts',(-16.6851208128819,-19.4847248545684,
-1.14131541449824));
#113158=CARTESIAN_POINT('Ctrl Pts',(-16.6871551199814,-19.4924951543287,
-1.14180287078307));
#113159=CARTESIAN_POINT('Ctrl Pts',(-16.6883007361917,-19.4968151025053,
-1.14207489622946));
#113160=CARTESIAN_POINT('Ctrl Pts',(-16.6917051437054,-19.50949048039,-1.14287599382586));
#113161=CARTESIAN_POINT('Ctrl Pts',(-16.6940014761971,-19.5178356057865,
-1.14340716516022));
#113162=CARTESIAN_POINT('Ctrl Pts',(-16.7104124668958,-19.576076357016,
-1.14713933633344));
#113163=CARTESIAN_POINT('Ctrl Pts',(-16.7263038615,-19.6254486306065,-1.1504320728655));
#113164=CARTESIAN_POINT('Ctrl Pts',(-16.7513457188333,-19.6944526689545,
-1.15517165026876));
#113165=CARTESIAN_POINT('Ctrl Pts',(-16.7590107151941,-19.7146081857888,
-1.15657311590473));
#113166=CARTESIAN_POINT('Ctrl Pts',(-16.7840719944143,-19.7775947722123,
-1.16099997778447));
#113167=CARTESIAN_POINT('Ctrl Pts',(-16.8025638202033,-19.8199746764711,
-1.16404776532646));
#113168=CARTESIAN_POINT('Ctrl Pts',(-16.8694205396727,-19.9604599662169,
-1.17432515973072));
#113169=CARTESIAN_POINT('Ctrl Pts',(-16.9239979012258,-20.0554237337135,
-1.18155611709649));
#113170=CARTESIAN_POINT('Ctrl Pts',(-17.0167265964488,-20.1912312064795,
-1.19212597824787));
#113171=CARTESIAN_POINT('Ctrl Pts',(-17.0495457919176,-20.2354861769175,
-1.19561326428979));
#113172=CARTESIAN_POINT('Ctrl Pts',(-17.1055411522579,-20.3051395539879,
-1.20116826928217));
#113173=CARTESIAN_POINT('Ctrl Pts',(-17.1276733761538,-20.3313403731348,
-1.2032743795307));
#113174=CARTESIAN_POINT('Ctrl Pts',(-17.1576060241161,-20.3650774337534,
-1.20601011230233));
#113175=CARTESIAN_POINT('Ctrl Pts',(-17.164840526552,-20.3731067358428,
-1.20666305704469));
#113176=CARTESIAN_POINT('Ctrl Pts',(-17.1767928496026,-20.3861696113741,
-1.20772850138904));
#113177=CARTESIAN_POINT('Ctrl Pts',(-17.1814742821618,-20.3912360753681,
-1.20814252985013));
#113178=CARTESIAN_POINT('Ctrl Pts',(-17.190585789053,-20.4010007832985,
-1.20894208165084));
#113179=CARTESIAN_POINT('Ctrl Pts',(-17.1950127547054,-20.4057018115139,
-1.20932773118715));
#113180=CARTESIAN_POINT('Ctrl Pts',(-17.2052865024455,-20.4165120509319,
-1.21021626879744));
#113181=CARTESIAN_POINT('Ctrl Pts',(-17.2111485424769,-20.4226066593126,
-1.21071849047337));
#113182=CARTESIAN_POINT('Ctrl Pts',(-17.2270173142075,-20.4389083686787,
-1.21206542043532));
#113183=CARTESIAN_POINT('Ctrl Pts',(-17.2370912734195,-20.4490496288815,
-1.21290718553109));
#113184=CARTESIAN_POINT('Ctrl Pts',(-17.3306416150942,-20.5413364240546,
-1.22060558191524));
#113185=CARTESIAN_POINT('Ctrl Pts',(-17.4207019398818,-20.6165295191162,
-1.22714391961088));
#113186=CARTESIAN_POINT('Ctrl Pts',(-17.6505928968053,-20.7781358035061,
-1.24252640308231));
#113187=CARTESIAN_POINT('Ctrl Pts',(-17.7951262372743,-20.8564806741519,
-1.25118391531412));
#113188=CARTESIAN_POINT('Ctrl Pts',(-17.976214436349,-20.9289737140594,
-1.26239998728148));
#113189=CARTESIAN_POINT('Ctrl Pts',(-18.0054548048088,-20.9399350321059,
-1.26422304119466));
#113190=CARTESIAN_POINT('Ctrl Pts',(-18.0416743067521,-20.952606223557,
-1.26650820836094));
#113191=CARTESIAN_POINT('Ctrl Pts',(-18.0484353456044,-20.9549331562959,
-1.26693592008741));
#113192=CARTESIAN_POINT('Ctrl Pts',(-18.0590822442749,-20.958537254408,
-1.26761144098931));
#113193=CARTESIAN_POINT('Ctrl Pts',(-18.0629603109275,-20.9598375097001,
-1.26785790775429));
#113194=CARTESIAN_POINT('Ctrl Pts',(-18.0702350407491,-20.9622531831667,
-1.26832106102532));
#113195=CARTESIAN_POINT('Ctrl Pts',(-18.0736307693733,-20.9633712387644,
-1.26853758948812));
#113196=CARTESIAN_POINT('Ctrl Pts',(-18.0814137343029,-20.965911973664,
-1.26903462827884));
#113197=CARTESIAN_POINT('Ctrl Pts',(-18.0858027851299,-20.9673289164672,
-1.26931547087678));
#113198=CARTESIAN_POINT('Ctrl Pts',(-18.0993957276365,-20.9716682078382,
-1.27018685796167));
#113199=CARTESIAN_POINT('Ctrl Pts',(-18.1086148598757,-20.9745418835357,
-1.2707801430648));
#113200=CARTESIAN_POINT('Ctrl Pts',(-18.2198831369804,-21.0083915995844,
-1.27796539504898));
#113201=CARTESIAN_POINT('Ctrl Pts',(-18.3241012098868,-21.031673084689,
-1.28493824032067));
#113202=CARTESIAN_POINT('Ctrl Pts',(-18.5378628955064,-21.0627307298022,
-1.29918768837418));
#113203=CARTESIAN_POINT('Ctrl Pts',(-18.6471743992129,-21.0700458188569,
-1.30644376519846));
#113204=CARTESIAN_POINT('Ctrl Pts',(-18.8191787198025,-21.0682122872552,
-1.31756380342891));
#113205=CARTESIAN_POINT('Ctrl Pts',(-18.8817356568463,-21.0647671917594,
-1.32154879729399));
#113206=CARTESIAN_POINT('Ctrl Pts',(-18.9688256643133,-21.0560831036814,
-1.32700389058882));
#113207=CARTESIAN_POINT('Ctrl Pts',(-18.9935538649445,-21.0531760214477,
-1.32854246982863));
#113208=CARTESIAN_POINT('Ctrl Pts',(-19.0367595567446,-21.0473222791134,
-1.33121315144019));
#113209=CARTESIAN_POINT('Ctrl Pts',(-19.0552595912429,-21.0445656770634,
-1.33235103508021));
#113210=CARTESIAN_POINT('Ctrl Pts',(-19.0821455865989,-21.0401945545604,
-1.33399688729359));
#113211=CARTESIAN_POINT('Ctrl Pts',(-19.0905617638768,-21.0387739597373,
-1.33451097206093));
#113212=CARTESIAN_POINT('Ctrl Pts',(-19.1053189390384,-21.0361911619444,
-1.33541048274113));
#113213=CARTESIAN_POINT('Ctrl Pts',(-19.1116636054813,-21.0350508290813,
-1.33579659809905));
#113214=CARTESIAN_POINT('Ctrl Pts',(-19.1239853952597,-21.0327780751215,
-1.33654529482105));
#113215=CARTESIAN_POINT('Ctrl Pts',(-19.1299630345564,-21.0316488364326,
-1.33690797330629));
#113216=CARTESIAN_POINT('Ctrl Pts',(-19.1442605975167,-21.0288839968661,
-1.33777420221956));
#113217=CARTESIAN_POINT('Ctrl Pts',(-19.1525757667027,-21.0272241385019,
-1.33827697549871));
#113218=CARTESIAN_POINT('Ctrl Pts',(-19.1826603130865,-21.0210305396005,
-1.34009255695913));
#113219=CARTESIAN_POINT('Ctrl Pts',(-19.2043683739302,-21.0162037443949,
-1.34139601175898));
#113220=CARTESIAN_POINT('Ctrl Pts',(-19.4052516317385,-20.9682036259441,
-1.35340673011112));
#113221=CARTESIAN_POINT('Ctrl Pts',(-19.5781414642451,-20.9021505404539,
-1.36327138102053));
#113222=CARTESIAN_POINT('Ctrl Pts',(-19.8115642434693,-20.7760352665265,
-1.37773074058416));
#113223=CARTESIAN_POINT('Ctrl Pts',(-19.8805508821496,-20.7334792654729,
-1.38218241140538));
#113224=CARTESIAN_POINT('Ctrl Pts',(-19.9766423679338,-20.6663056014761,
-1.38888719238138));
#113225=CARTESIAN_POINT('Ctrl Pts',(-20.0058197935248,-20.6447722256088,
-1.39099590238403));
#113226=CARTESIAN_POINT('Ctrl Pts',(-20.0403302873196,-20.6179069994832,
-1.39359851447107));
#113227=CARTESIAN_POINT('Ctrl Pts',(-20.0462081858515,-20.6132810188803,
-1.3940457013601));
#113228=CARTESIAN_POINT('Ctrl Pts',(-20.0553184713441,-20.6060325939564,
-1.3947451250928));
#113229=CARTESIAN_POINT('Ctrl Pts',(-20.0585679151092,-20.6034315493424,
-1.39499585701764));
#113230=CARTESIAN_POINT('Ctrl Pts',(-20.0645866491574,-20.5985846112994,
-1.39546266537871));
#113231=CARTESIAN_POINT('Ctrl Pts',(-20.0673579438965,-20.596341298493,
-1.39567855713391));
#113232=CARTESIAN_POINT('Ctrl Pts',(-20.0736190033552,-20.5912468493669,
-1.39616846621913));
#113233=CARTESIAN_POINT('Ctrl Pts',(-20.0771053215513,-20.5883915795621,
-1.39644277966131));
#113234=CARTESIAN_POINT('Ctrl Pts',(-20.0873944805958,-20.5799097998947,
-1.39725679905749));
#113235=CARTESIAN_POINT('Ctrl Pts',(-20.0941711743339,-20.574251924635,
-1.39779870495772));
#113236=CARTESIAN_POINT('Ctrl Pts',(-20.1437897748362,-20.5322957920663,
-1.40180794424738));
#113237=CARTESIAN_POINT('Ctrl Pts',(-20.1852040735271,-20.4943513057331,
-1.40538276734724));
#113238=CARTESIAN_POINT('Ctrl Pts',(-20.2694068852616,-20.4108069874383,
-1.41306245080667));
#113239=CARTESIAN_POINT('Ctrl Pts',(-20.3117851875953,-20.3648642600338,
-1.41717770387232));
#113240=CARTESIAN_POINT('Ctrl Pts',(-20.4227519314223,-20.2333357899058,
-1.4285446052632));
#113241=CARTESIAN_POINT('Ctrl Pts',(-20.4868273204476,-20.1441846905486,
-1.43579421479988));
#113242=CARTESIAN_POINT('Ctrl Pts',(-20.5724489213871,-20.0031240137737,
-1.44640321064745));
#113243=CARTESIAN_POINT('Ctrl Pts',(-20.5993182410521,-19.9546688492893,
-1.4499108553119));
#113244=CARTESIAN_POINT('Ctrl Pts',(-20.6397608422569,-19.8744695415408,
-1.45549443177426));
#113245=CARTESIAN_POINT('Ctrl Pts',(-20.6545119772732,-19.8433520106125,
-1.45760925332541));
#113246=CARTESIAN_POINT('Ctrl Pts',(-20.6728942833821,-19.8019971136178,
-1.46035443784606));
#113247=CARTESIAN_POINT('Ctrl Pts',(-20.6772145078748,-19.7920735196925,
-1.46100832781741));
#113248=CARTESIAN_POINT('Ctrl Pts',(-20.6841645660995,-19.7757686510845,
-1.46207489748118));
#113249=CARTESIAN_POINT('Ctrl Pts',(-20.6868395938445,-19.7694069658667,
-1.46248911262404));
#113250=CARTESIAN_POINT('Ctrl Pts',(-20.6919565604378,-19.7570694248642,
-1.4632887369795));
#113251=CARTESIAN_POINT('Ctrl Pts',(-20.6944023645908,-19.7510952644985,
-1.46367427388952));
#113252=CARTESIAN_POINT('Ctrl Pts',(-20.6999852470215,-19.7372785196961,
-1.46456214063773));
#113253=CARTESIAN_POINT('Ctrl Pts',(-20.7031028045932,-19.7294281272891,
-1.46506380701488));
#113254=CARTESIAN_POINT('Ctrl Pts',(-20.7113578717422,-19.7082726095752,
-1.46640833455584));
#113255=CARTESIAN_POINT('Ctrl Pts',(-20.7164081053056,-19.6949337331012,
-1.46724826858965));
#113256=CARTESIAN_POINT('Ctrl Pts',(-20.7217433569485,-19.6804001874366,
-1.46815528110785));
#113257=CARTESIAN_POINT('Ctrl Pts',(-20.72216246852,-19.6792554467231,-1.46822666771441));
#113258=CARTESIAN_POINT('Ctrl Pts',(-20.7225805819607,-19.6781103697434,
-1.46829802089257));
#113259=CARTESIAN_POINT('',(-20.8509993841888,-18.9503852727442,-0.489056278967187));
#113260=CARTESIAN_POINT('Ctrl Pts',(-20.7225806439552,-19.6781101999604,
-1.24458624895942));
#113261=CARTESIAN_POINT('Ctrl Pts',(-20.6661823420556,-19.8325668809376,
-1.23372063291377));
#113262=CARTESIAN_POINT('Ctrl Pts',(-20.5919347480107,-19.9800493809754,
-1.22298087846725));
#113263=CARTESIAN_POINT('Ctrl Pts',(-20.4894885518365,-20.1353879489779,
-1.21154553712518));
#113264=CARTESIAN_POINT('Ctrl Pts',(-20.4774343962679,-20.1530760392754,
-1.21024031609317));
#113265=CARTESIAN_POINT('Ctrl Pts',(-20.4603098215144,-20.1774032193866,
-1.20844026140752));
#113266=CARTESIAN_POINT('Ctrl Pts',(-20.4554655649895,-20.1841992377921,
-1.20793685243739));
#113267=CARTESIAN_POINT('Ctrl Pts',(-20.4470413923941,-20.1958708819646,
-1.20707127883651));
#113268=CARTESIAN_POINT('Ctrl Pts',(-20.4434805626339,-20.2007601011453,
-1.20670838439107));
#113269=CARTESIAN_POINT('Ctrl Pts',(-20.4360698922163,-20.2108442672094,
-1.20595923331404));
#113270=CARTESIAN_POINT('Ctrl Pts',(-20.4322171031056,-20.2160369770011,
-1.20557309651764));
#113271=CARTESIAN_POINT('Ctrl Pts',(-20.4231495686122,-20.2281417249901,
-1.20467205338959));
#113272=CARTESIAN_POINT('Ctrl Pts',(-20.4179160645021,-20.2350396168909,
-1.20415788796871));
#113273=CARTESIAN_POINT('Ctrl Pts',(-20.400833264236,-20.2572706114968,
-1.20249833136461));
#113274=CARTESIAN_POINT('Ctrl Pts',(-20.3888155115931,-20.272473460348,
-1.20135960267726));
#113275=CARTESIAN_POINT('Ctrl Pts',(-20.3265596928535,-20.349044093152,
-1.19560095950256));
#113276=CARTESIAN_POINT('Ctrl Pts',(-20.2731077263145,-20.4077224817765,
-1.19111364917385));
#113277=CARTESIAN_POINT('Ctrl Pts',(-20.1000687157715,-20.5774657606864,
-1.17766510614145));
#113278=CARTESIAN_POINT('Ctrl Pts',(-19.9708583561275,-20.6778210692345,
-1.16906408067147));
#113279=CARTESIAN_POINT('Ctrl Pts',(-19.7791772409136,-20.794016751747,
-1.15653482464692));
#113280=CARTESIAN_POINT('Ctrl Pts',(-19.7255935645414,-20.823406400002,
-1.15304837588591));
#113281=CARTESIAN_POINT('Ctrl Pts',(-19.6626470098079,-20.8544686056655,
-1.14888521636218));
#113282=CARTESIAN_POINT('Ctrl Pts',(-19.6544481996829,-20.8584488373225,
-1.14834167811425));
#113283=CARTESIAN_POINT('Ctrl Pts',(-19.6421585445052,-20.8643172738121,
-1.14752464758654));
#113284=CARTESIAN_POINT('Ctrl Pts',(-19.6380868334741,-20.8662456201739,
-1.1472535820609));
#113285=CARTESIAN_POINT('Ctrl Pts',(-19.6307806854683,-20.8696772730928,
-1.14676646819602));
#113286=CARTESIAN_POINT('Ctrl Pts',(-19.6275485790196,-20.8711854152749,
-1.14655072293413));
#113287=CARTESIAN_POINT('Ctrl Pts',(-19.6205324434656,-20.8744376679082,
-1.14608182704168));
#113288=CARTESIAN_POINT('Ctrl Pts',(-19.6167471219066,-20.8761787542702,
-1.14582850047923));
#113289=CARTESIAN_POINT('Ctrl Pts',(-19.6061408201004,-20.8810193163291,
-1.14511776581438));
#113290=CARTESIAN_POINT('Ctrl Pts',(-19.599308568291,-20.8840937375409,
-1.14465886514953));
#113291=CARTESIAN_POINT('Ctrl Pts',(-19.5591795902109,-20.9018956946936,
-1.14195791219407));
#113292=CARTESIAN_POINT('Ctrl Pts',(-19.5255258327402,-20.9157976128018,
-1.13967026937973));
#113293=CARTESIAN_POINT('Ctrl Pts',(-19.4153871114746,-20.9580035462417,
-1.13214930869362));
#113294=CARTESIAN_POINT('Ctrl Pts',(-19.3376238590628,-20.9827572731476,
-1.12678916334));
#113295=CARTESIAN_POINT('Ctrl Pts',(-19.0810907958565,-21.0483779830773,
-1.10930511712457));
#113296=CARTESIAN_POINT('Ctrl Pts',(-18.8983629554454,-21.0705570774497,
-1.09724052908153));
#113297=CARTESIAN_POINT('Ctrl Pts',(-18.692724930536,-21.0687152236704,
-1.08459113297433));
#113298=CARTESIAN_POINT('Ctrl Pts',(-18.6704145147232,-21.0681625446401,
-1.08322946316258));
#113299=CARTESIAN_POINT('Ctrl Pts',(-18.6396301016288,-21.0669126357501,
-1.08136476141177));
#113300=CARTESIAN_POINT('Ctrl Pts',(-18.63114594162,-21.0665170088076,-1.0808523346566));
#113301=CARTESIAN_POINT('Ctrl Pts',(-18.6165841428066,-21.0657501241288,
-1.07997531686111));
#113302=CARTESIAN_POINT('Ctrl Pts',(-18.6105053522402,-21.0654036869358,
-1.07960995208983));
#113303=CARTESIAN_POINT('Ctrl Pts',(-18.597992781016,-21.0646364110564,
-1.0788593880015));
#113304=CARTESIAN_POINT('Ctrl Pts',(-18.5915592531782,-21.0642123955703,
-1.07847429238584));
#113305=CARTESIAN_POINT('Ctrl Pts',(-18.5766197305293,-21.0631592067378,
-1.07758190379666));
#113306=CARTESIAN_POINT('Ctrl Pts',(-18.5681153629804,-21.0625080042162,
-1.07707530749062));
#113307=CARTESIAN_POINT('Ctrl Pts',(-18.5410186473279,-21.0602683384612,
-1.07546548286585));
#113308=CARTESIAN_POINT('Ctrl Pts',(-18.5224429415029,-21.0584854220796,
-1.07436835997421));
#113309=CARTESIAN_POINT('Ctrl Pts',(-18.3441735034812,-21.0389929439099,
-1.06389553117215));
#113310=CARTESIAN_POINT('Ctrl Pts',(-18.1869583414912,-21.003403869076,
-1.05514828860677));
#113311=CARTESIAN_POINT('Ctrl Pts',(-17.9084935426492,-20.9060379886269,
-1.03912854452344));
#113312=CARTESIAN_POINT('Ctrl Pts',(-17.7862426480781,-20.8497543200834,
-1.03186589658319));
#113313=CARTESIAN_POINT('Ctrl Pts',(-17.656607916401,-20.7744053181977,
-1.02307442102728));
#113314=CARTESIAN_POINT('Ctrl Pts',(-17.6431403977316,-20.7663759646988,
-1.02214690228698));
#113315=CARTESIAN_POINT('Ctrl Pts',(-17.6248246333446,-20.7551784489659,
-1.02086417720725));
#113316=CARTESIAN_POINT('Ctrl Pts',(-17.6198979818765,-20.7521386625013,
-1.02051700874684));
#113317=CARTESIAN_POINT('Ctrl Pts',(-17.6120883109699,-20.747275688475,
-1.01996317633543));
#113318=CARTESIAN_POINT('Ctrl Pts',(-17.6091970814683,-20.7454656477596,
-1.0197573735147));
#113319=CARTESIAN_POINT('Ctrl Pts',(-17.6032371940535,-20.7417144078601,
-1.01933152364533));
#113320=CARTESIAN_POINT('Ctrl Pts',(-17.6001691636093,-20.7397723061611,
-1.01911141362441));
#113321=CARTESIAN_POINT('Ctrl Pts',(-17.5928705319652,-20.7351258365693,
-1.01858568352044));
#113322=CARTESIAN_POINT('Ctrl Pts',(-17.5886445411204,-20.7324143010771,
-1.01827959036972));
#113323=CARTESIAN_POINT('Ctrl Pts',(-17.5744204527725,-20.7232160550712,
-1.01724372036873));
#113324=CARTESIAN_POINT('Ctrl Pts',(-17.5644677098496,-20.7166600940052,
-1.01650953184276));
#113325=CARTESIAN_POINT('Ctrl Pts',(-17.540689410603,-20.7007076003327,
-1.01473383048842));
#113326=CARTESIAN_POINT('Ctrl Pts',(-17.5269189469453,-20.6912307865022,
-1.01368767159871));
#113327=CARTESIAN_POINT('Ctrl Pts',(-17.4756948782964,-20.6550770995942,
-1.00973304630827));
#113328=CARTESIAN_POINT('Ctrl Pts',(-17.4390033230139,-20.6273466648571,
-1.00677227010053));
#113329=CARTESIAN_POINT('Ctrl Pts',(-17.3454270830285,-20.5517128670429,
-0.998935716966504));
#113330=CARTESIAN_POINT('Ctrl Pts',(-17.2901113344371,-20.5019680554739,
-0.99401212471712));
#113331=CARTESIAN_POINT('Ctrl Pts',(-17.1277266796459,-20.3396860537082,
-0.978845205443246));
#113332=CARTESIAN_POINT('Ctrl Pts',(-17.0303087573192,-20.2181908556132,
-0.968729374174171));
#113333=CARTESIAN_POINT('Ctrl Pts',(-16.9342096071964,-20.0669065472817,
-0.957687408827122));
#113334=CARTESIAN_POINT('Ctrl Pts',(-16.9217171354024,-20.0464829645925,
-0.956225145876773));
#113335=CARTESIAN_POINT('Ctrl Pts',(-16.9046537474558,-20.0174930080576,
-0.954188309082515));
#113336=CARTESIAN_POINT('Ctrl Pts',(-16.8997915754078,-20.0091009989466,
-0.953603162011575));
#113337=CARTESIAN_POINT('Ctrl Pts',(-16.8920196450153,-19.9954717341781,
-0.952659964534795));
#113338=CARTESIAN_POINT('Ctrl Pts',(-16.8890741879184,-19.9902550925667,
-0.952300626726747));
#113339=CARTESIAN_POINT('Ctrl Pts',(-16.8829819345063,-19.979357433358,
-0.951553413427386));
#113340=CARTESIAN_POINT('Ctrl Pts',(-16.8798390522542,-19.9736742905474,
-0.951165681462966));
#113341=CARTESIAN_POINT('Ctrl Pts',(-16.8724721964518,-19.9602071546126,
-0.950251414745203));
#113342=CARTESIAN_POINT('Ctrl Pts',(-16.8682707964321,-19.9524109018718,
-0.949725690312238));
#113343=CARTESIAN_POINT('Ctrl Pts',(-16.8544956832457,-19.9264607394634,
-0.947987351125742));
#113344=CARTESIAN_POINT('Ctrl Pts',(-16.8451368537631,-19.9081936351888,
-0.946782341173989));
#113345=CARTESIAN_POINT('Ctrl Pts',(-16.7969202976145,-19.810610399808,
-0.940438829375276));
#113346=CARTESIAN_POINT('Ctrl Pts',(-16.7627867205766,-19.7290523564093,
-0.935466793701247));
#113347=CARTESIAN_POINT('Ctrl Pts',(-16.6909632089416,-19.5219305385132,
-0.923366387270467));
#113348=CARTESIAN_POINT('Ctrl Pts',(-16.6596431278252,-19.3945632604551,
-0.916389198105422));
#113349=CARTESIAN_POINT('Ctrl Pts',(-16.6347059999534,-19.2278193987965,
-0.907089195435979));
#113350=CARTESIAN_POINT('Ctrl Pts',(-16.6301253420164,-19.1903754013159,
-0.904988791609812));
#113351=CARTESIAN_POINT('Ctrl Pts',(-16.6221957050251,-19.1071643358583,
-0.900257140621528));
#113352=CARTESIAN_POINT('Ctrl Pts',(-16.6193297205363,-19.0613722280543,
-0.89761064508369));
#113353=CARTESIAN_POINT('Ctrl Pts',(-16.6177244937089,-19.007903114256,
-0.894433887255013));
#113354=CARTESIAN_POINT('Ctrl Pts',(-16.6175368194285,-19.0002781319863,
-0.893978812199759));
#113355=CARTESIAN_POINT('Ctrl Pts',(-16.6173018872752,-18.9880461539762,
-0.893245253663853));
#113356=CARTESIAN_POINT('Ctrl Pts',(-16.617228455125,-18.9834396488026,
-0.892968196487284));
#113357=CARTESIAN_POINT('Ctrl Pts',(-16.61712466768,-18.9752519527732,-0.892474265397267));
#113358=CARTESIAN_POINT('Ctrl Pts',(-16.6170883622654,-18.9716708852444,
-0.892257727461891));
#113359=CARTESIAN_POINT('Ctrl Pts',(-16.6170304186042,-18.9640471715229,
-0.891795644351456));
#113360=CARTESIAN_POINT('Ctrl Pts',(-16.6170112734264,-18.9600046126915,
-0.891549968274009));
#113361=CARTESIAN_POINT('Ctrl Pts',(-16.6169907237584,-18.9490245829682,
-0.890880961851548));
#113362=CARTESIAN_POINT('Ctrl Pts',(-16.6170118418035,-18.9420871912966,
-0.890456402181877));
#113363=CARTESIAN_POINT('Ctrl Pts',(-16.617293210134,-18.9067374667283,
-0.888283951342084));
#113364=CARTESIAN_POINT('Ctrl Pts',(-16.618091344353,-18.8783338039578,
-0.886508468251654));
#113365=CARTESIAN_POINT('Ctrl Pts',(-16.6221157620144,-18.7949400759451,
-0.881224236880963));
#113366=CARTESIAN_POINT('Ctrl Pts',(-16.6269167083662,-18.7400518345294,
-0.877655291514327));
#113367=CARTESIAN_POINT('Ctrl Pts',(-16.65147202781,-18.5466041013743,-0.864884454562608));
#113368=CARTESIAN_POINT('Ctrl Pts',(-16.6828138324906,-18.4098663781984,
-0.855532658905493));
#113369=CARTESIAN_POINT('Ctrl Pts',(-16.7562374772549,-18.1915276702295,
-0.840658450403927));
#113370=CARTESIAN_POINT('Ctrl Pts',(-16.7905171998272,-18.1077600411421,
-0.834959681366878));
#113371=CARTESIAN_POINT('Ctrl Pts',(-16.836057805489,-18.0140804844457,
-0.828604027268443));
#113372=CARTESIAN_POINT('Ctrl Pts',(-16.8421820600796,-18.0017881880842,
-0.827770278962194));
#113373=CARTESIAN_POINT('Ctrl Pts',(-16.8521963996708,-17.9821685689714,
-0.826439688166557));
#113374=CARTESIAN_POINT('Ctrl Pts',(-16.8560106148612,-17.9748031584242,
-0.825940203278252));
#113375=CARTESIAN_POINT('Ctrl Pts',(-16.8628603671227,-17.9617642336197,
-0.82505596551924));
#113376=CARTESIAN_POINT('Ctrl Pts',(-16.8658786504242,-17.9560818189135,
-0.824670609817944));
#113377=CARTESIAN_POINT('Ctrl Pts',(-16.872221887875,-17.9442699345436,
-0.823869539515819));
#113378=CARTESIAN_POINT('Ctrl Pts',(-16.8755513185703,-17.9381429470129,
-0.823453989786786));
#113379=CARTESIAN_POINT('Ctrl Pts',(-16.8842775647081,-17.9222718896201,
-0.822377440304785));
#113380=CARTESIAN_POINT('Ctrl Pts',(-16.889721162235,-17.912553683605,-0.821718118394523));
#113381=CARTESIAN_POINT('Ctrl Pts',(-16.9137064766448,-17.8705154483635,
-0.818865000877634));
#113382=CARTESIAN_POINT('Ctrl Pts',(-16.9330236198484,-17.838643958865,
-0.816699273047077));
#113383=CARTESIAN_POINT('Ctrl Pts',(-16.9865971554088,-17.7552989840656,
-0.811013087269197));
#113384=CARTESIAN_POINT('Ctrl Pts',(-17.0222843534298,-17.7047869361817,
-0.807543773668025));
#113385=CARTESIAN_POINT('Ctrl Pts',(-17.1467956067731,-17.5439843609605,
-0.796291847144478));
#113386=CARTESIAN_POINT('Ctrl Pts',(-17.2444599190256,-17.4410420768077,
-0.788767944894847));
#113387=CARTESIAN_POINT('Ctrl Pts',(-17.4090573587147,-17.2991362216952,
-0.776737456263016));
#113388=CARTESIAN_POINT('Ctrl Pts',(-17.4690615245864,-17.2527767252116,
-0.772455925017883));
#113389=CARTESIAN_POINT('Ctrl Pts',(-17.5392389823377,-17.2043371262278,
-0.767402312202162));
#113390=CARTESIAN_POINT('Ctrl Pts',(-17.5471004002235,-17.1989886645767,
-0.766835563151585));
#113391=CARTESIAN_POINT('Ctrl Pts',(-17.558807110148,-17.1911389290952,
-0.765990239723609));
#113392=CARTESIAN_POINT('Ctrl Pts',(-17.5626250568805,-17.1885968183335,
-0.765714339488015));
#113393=CARTESIAN_POINT('Ctrl Pts',(-17.5694381726738,-17.1840923179106,
-0.765221562130502));
#113394=CARTESIAN_POINT('Ctrl Pts',(-17.5724300862887,-17.1821251012263,
-0.765005012789305));
#113395=CARTESIAN_POINT('Ctrl Pts',(-17.5788826676815,-17.1779058661085,
-0.764537650669552));
#113396=CARTESIAN_POINT('Ctrl Pts',(-17.5823448928539,-17.1756564068724,
-0.764286678873976));
#113397=CARTESIAN_POINT('Ctrl Pts',(-17.591928511475,-17.1694695823861,
-0.763591468520061));
#113398=CARTESIAN_POINT('Ctrl Pts',(-17.5980635966468,-17.1655536787713,
-0.763145850445403));
#113399=CARTESIAN_POINT('Ctrl Pts',(-17.6319409930451,-17.1441754741181,
-0.760682597581648));
#113400=CARTESIAN_POINT('Ctrl Pts',(-17.6600642134983,-17.1273287352435,
-0.758628267009439));
#113401=CARTESIAN_POINT('Ctrl Pts',(-17.8308812954873,-17.030320612999,
-0.746145962448446));
#113402=CARTESIAN_POINT('Ctrl Pts',(-17.9820855660748,-16.9662759372,-0.735128700240828));
#113403=CARTESIAN_POINT('Ctrl Pts',(-18.2489533329964,-16.8881426260486,
-0.716988446011342));
#113404=CARTESIAN_POINT('Ctrl Pts',(-18.3611876309905,-16.8649456676826,
-0.70970887755997));
#113405=CARTESIAN_POINT('Ctrl Pts',(-18.4889228391326,-16.8491852852282,
-0.701850727411099));
#113406=CARTESIAN_POINT('Ctrl Pts',(-18.5030997550142,-16.8475814028804,
-0.700984159919865));
#113407=CARTESIAN_POINT('Ctrl Pts',(-18.5257061175593,-16.8452550689986,
-0.699611003539678));
#113408=CARTESIAN_POINT('Ctrl Pts',(-18.5341253637235,-16.8444396381666,
-0.699101510074506));
#113409=CARTESIAN_POINT('Ctrl Pts',(-18.5489929004768,-16.8430895622128,
-0.698205098472977));
#113410=CARTESIAN_POINT('Ctrl Pts',(-18.5554391366547,-16.8425339820225,
-0.697817528159776));
#113411=CARTESIAN_POINT('Ctrl Pts',(-18.5687874047758,-16.8414451633194,
-0.697017208627248));
#113412=CARTESIAN_POINT('Ctrl Pts',(-18.575689715888,-16.8409162082126,
-0.696604598181632));
#113413=CARTESIAN_POINT('Ctrl Pts',(-18.5934351201831,-16.8396438187476,
-0.695546898181894));
#113414=CARTESIAN_POINT('Ctrl Pts',(-18.6042816533274,-16.838950005536,
-0.694903368007642));
#113415=CARTESIAN_POINT('Ctrl Pts',(-18.6497600393507,-16.8363924185133,
-0.692217084498543));
#113416=CARTESIAN_POINT('Ctrl Pts',(-18.6844308352284,-16.8352962157233,
-0.6901983668217));
#113417=CARTESIAN_POINT('Ctrl Pts',(-18.7749975637378,-16.8346593857365,
-0.68498914065463));
#113418=CARTESIAN_POINT('Ctrl Pts',(-18.8308768709355,-16.8364793507137,
-0.681839231688125));
#113419=CARTESIAN_POINT('Ctrl Pts',(-19.0845520339329,-16.8548153909185,
-0.667705195157753));
#113420=CARTESIAN_POINT('Ctrl Pts',(-19.2794561841048,-16.8968775714436,
-0.657394736191735));
#113421=CARTESIAN_POINT('Ctrl Pts',(-19.4955716737775,-16.9764707687702,
-0.644170640165188));
#113422=CARTESIAN_POINT('Ctrl Pts',(-19.5252592060564,-16.9881731796752,
-0.642310073980115));
#113423=CARTESIAN_POINT('Ctrl Pts',(-19.5609544653769,-17.003184512385,
-0.640006136709419));
#113424=CARTESIAN_POINT('Ctrl Pts',(-19.5672269241438,-17.0058580774774,
-0.639598742980857));
#113425=CARTESIAN_POINT('Ctrl Pts',(-19.5775381800859,-17.0103121208054,
-0.638924664551405));
#113426=CARTESIAN_POINT('Ctrl Pts',(-19.5815845733286,-17.0120750345136,
-0.638659026358655));
#113427=CARTESIAN_POINT('Ctrl Pts',(-19.5888755231298,-17.0152786873457,
-0.638178326549731));
#113428=CARTESIAN_POINT('Ctrl Pts',(-19.5921219984902,-17.0167149464509,
-0.637963541108073));
#113429=CARTESIAN_POINT('Ctrl Pts',(-19.5984335811427,-17.0195262307363,
-0.637544504456728));
#113430=CARTESIAN_POINT('Ctrl Pts',(-19.6014989849624,-17.0209003661585,
-0.637340315752203));
#113431=CARTESIAN_POINT('Ctrl Pts',(-19.6105425853905,-17.0249802398308,
-0.636735959008615));
#113432=CARTESIAN_POINT('Ctrl Pts',(-19.6165114206642,-17.0277064543452,
-0.636334549578813));
#113433=CARTESIAN_POINT('Ctrl Pts',(-19.6448671951683,-17.0408173890174,
-0.63441587118083));
#113434=CARTESIAN_POINT('Ctrl Pts',(-19.6670830653751,-17.0515648159411,
-0.632877741802317));
#113435=CARTESIAN_POINT('Ctrl Pts',(-19.72928114307,-17.0830079997259,-0.628482572726861));
#113436=CARTESIAN_POINT('Ctrl Pts',(-19.7687968860003,-17.1045935662158,
-0.625584773412187));
#113437=CARTESIAN_POINT('Ctrl Pts',(-19.8895209047652,-17.1756281997965,
-0.616463024098987));
#113438=CARTESIAN_POINT('Ctrl Pts',(-19.9681082336591,-17.229298158072,
-0.610137882435616));
#113439=CARTESIAN_POINT('Ctrl Pts',(-20.1606326761606,-17.380734559692,
-0.593981586666354));
#113440=CARTESIAN_POINT('Ctrl Pts',(-20.2682887424195,-17.4856678468788,
-0.584307120692968));
#113441=CARTESIAN_POINT('Ctrl Pts',(-20.3729857366812,-17.6119946244293,
-0.574291013654049));
#113442=CARTESIAN_POINT('Ctrl Pts',(-20.3818931718843,-17.6229639730383,
-0.573432898024258));
#113443=CARTESIAN_POINT('Ctrl Pts',(-20.3959063681158,-17.6405784736316,
-0.572073073340814));
#113444=CARTESIAN_POINT('Ctrl Pts',(-20.4010835361085,-17.6471660323951,
-0.571568488046995));
#113445=CARTESIAN_POINT('Ctrl Pts',(-20.4101514297626,-17.6588463148458,
-0.570680724869194));
#113446=CARTESIAN_POINT('Ctrl Pts',(-20.4140583677801,-17.6639262632966,
-0.5702969011356));
#113447=CARTESIAN_POINT('Ctrl Pts',(-20.422097144815,-17.6744773843779,
-0.569504357168962));
#113448=CARTESIAN_POINT('Ctrl Pts',(-20.4262255985482,-17.6799510508288,
-0.569095773986404));
#113449=CARTESIAN_POINT('Ctrl Pts',(-20.43676584734,-17.6940678552726,-0.568048536260453));
#113450=CARTESIAN_POINT('Ctrl Pts',(-20.4431385100698,-17.7027400704754,
-0.56741142291253));
#113451=CARTESIAN_POINT('Ctrl Pts',(-20.4695464598245,-17.7392575584162,
-0.5647540918308));
#113452=CARTESIAN_POINT('Ctrl Pts',(-20.4889702401525,-17.7675400396342,
-0.562757567744567));
#113453=CARTESIAN_POINT('Ctrl Pts',(-20.5378433424859,-17.8425464601744,
-0.557608819686927));
#113454=CARTESIAN_POINT('Ctrl Pts',(-20.5661675725709,-17.8899733527495,
-0.554496467580978));
#113455=CARTESIAN_POINT('Ctrl Pts',(-20.6274486114797,-18.0023487122949,
-0.547383506223037));
#113456=CARTESIAN_POINT('Ctrl Pts',(-20.6589739959099,-18.067997180263,
-0.543420718962677));
#113457=CARTESIAN_POINT('Ctrl Pts',(-20.7006448004888,-18.1676293066662,
-0.537557147698845));
#113458=CARTESIAN_POINT('Ctrl Pts',(-20.7134202568039,-18.2004518733808,
-0.535648298079368));
#113459=CARTESIAN_POINT('Ctrl Pts',(-20.7392639646576,-18.272087190512,
-0.531505618451721));
#113460=CARTESIAN_POINT('Ctrl Pts',(-20.7520366525749,-18.3109907112703,
-0.529270323297309));
#113461=CARTESIAN_POINT('Ctrl Pts',(-20.7690499488225,-18.368374677458,
-0.52596440823563));
#113462=CARTESIAN_POINT('Ctrl Pts',(-20.7741834180245,-18.3865812122226,
-0.5249142252036));
#113463=CARTESIAN_POINT('Ctrl Pts',(-20.7947008200014,-18.4632692387766,
-0.52047639537556));
#113464=CARTESIAN_POINT('Ctrl Pts',(-20.8078179693683,-18.5223219603253,
-0.517024578340226));
#113465=CARTESIAN_POINT('Ctrl Pts',(-20.8199725808871,-18.5907667919248,
-0.512901088674033));
#113466=CARTESIAN_POINT('Ctrl Pts',(-20.8214989814923,-18.5996946857741,
-0.512360842528588));
#113467=CARTESIAN_POINT('Ctrl Pts',(-20.8236943601964,-18.6130508365701,
-0.511548707398552));
#113468=CARTESIAN_POINT('Ctrl Pts',(-20.8244066763095,-18.6174720023458,
-0.511279232147322));
#113469=CARTESIAN_POINT('Ctrl Pts',(-20.8256596119144,-18.6254089394062,
-0.510794262174948));
#113470=CARTESIAN_POINT('Ctrl Pts',(-20.8262054025299,-18.628923838553,
-0.510579064774684));
#113471=CARTESIAN_POINT('Ctrl Pts',(-20.827252039116,-18.6357780801854,
-0.510158586227158));
#113472=CARTESIAN_POINT('Ctrl Pts',(-20.8277537529317,-18.6391172367318,
-0.509953361381815));
#113473=CARTESIAN_POINT('Ctrl Pts',(-20.8288494962056,-18.6465306225135,
-0.509496908631086));
#113474=CARTESIAN_POINT('Ctrl Pts',(-20.8294396311101,-18.6506054014143,
-0.509245465875732));
#113475=CARTESIAN_POINT('Ctrl Pts',(-20.8308795002836,-18.6607561149897,
-0.508617762711576));
#113476=CARTESIAN_POINT('Ctrl Pts',(-20.831714710083,-18.6668340267681,
-0.508240727451475));
#113477=CARTESIAN_POINT('Ctrl Pts',(-20.8356021821279,-18.6960651320066,
-0.506421988151926));
#113478=CARTESIAN_POINT('Ctrl Pts',(-20.8382974724732,-18.7192631654612,
-0.504962284114994));
#113479=CARTESIAN_POINT('Ctrl Pts',(-20.8474812861682,-18.8116101392643,
-0.499099022991545));
#113480=CARTESIAN_POINT('Ctrl Pts',(-20.8509485264066,-18.8810102963083,
-0.494577353553003));
#113481=CARTESIAN_POINT('Ctrl Pts',(-20.8509994311265,-18.9504480302427,
-0.490010487033197));
#113482=CARTESIAN_POINT('Ctrl Pts',(-20.8509993841888,-18.9503852727442,
-0.489056278967187));
#113483=CARTESIAN_POINT('Ctrl Pts',(-20.8510540303841,-19.0220295465461,
-0.484732818461429));
#113484=CARTESIAN_POINT('Ctrl Pts',(-20.847467542629,-19.0938083387668,
-0.480409357955671));
#113485=CARTESIAN_POINT('Ctrl Pts',(-20.8402254594309,-19.1653150581775,
-0.476085897449914));
#113486=CARTESIAN_POINT('Ctrl Pts',(-20.832990974746,-19.2367467515573,
-0.471766973190315));
#113487=CARTESIAN_POINT('Ctrl Pts',(-20.8221085463431,-19.3079064470899,
-0.467448048930716));
#113488=CARTESIAN_POINT('Ctrl Pts',(-20.8076157348804,-19.3783880674413,
-0.463129124671117));
#113489=CARTESIAN_POINT('Ctrl Pts',(-20.7931333507106,-19.4488189776526,
-0.458813307792603));
#113490=CARTESIAN_POINT('Ctrl Pts',(-20.7750458355094,-19.518572295312,
-0.45449749091409));
#113491=CARTESIAN_POINT('Ctrl Pts',(-20.7534422763271,-19.5872494727135,
-0.450181674035576));
#113492=CARTESIAN_POINT('Ctrl Pts',(-20.7438446524082,-19.6177600804772,
-0.448264323891871));
#113493=CARTESIAN_POINT('Ctrl Pts',(-20.7335537498538,-19.6480584251371,
-0.446346973748166));
#113494=CARTESIAN_POINT('Ctrl Pts',(-20.7225805821191,-19.6781103693095,
-0.444429623604461));
#113495=CARTESIAN_POINT('Origin',(-23.734,10.1295,-7.));
#113496=CARTESIAN_POINT('',(-20.7043183293681,10.1259540182473,-11.2629985252183));
#113497=CARTESIAN_POINT('Ctrl Pts',(-22.1191569086782,11.6181146495903,
-10.9946458447559));
#113498=CARTESIAN_POINT('Ctrl Pts',(-22.1119092629397,11.7394000803016,
-10.9494485291601));
#113499=CARTESIAN_POINT('Ctrl Pts',(-22.1046616172012,11.8586337142555,
-10.8987204065082));
#113500=CARTESIAN_POINT('Ctrl Pts',(-22.0974139714626,11.975312836413,-10.8426740654046));
#113501=CARTESIAN_POINT('Ctrl Pts',(-22.0901668807576,12.0919830231423,
-10.7866320163975));
#113502=CARTESIAN_POINT('Ctrl Pts',(-22.0829197900526,12.2060987775499,
-10.7252727140119));
#113503=CARTESIAN_POINT('Ctrl Pts',(-22.0756726993475,12.3171800739265,
-10.6588556809671));
#113504=CARTESIAN_POINT('Ctrl Pts',(-22.0684238466281,12.4282883779462,
-10.5924224996814));
#113505=CARTESIAN_POINT('Ctrl Pts',(-22.0611749939087,12.5363604522096,
-10.5209293079317));
#113506=CARTESIAN_POINT('Ctrl Pts',(-22.0539261411893,12.6409430705206,
-10.4446803485279));
#113507=CARTESIAN_POINT('Ctrl Pts',(-22.0488803813273,12.7137406287231,
-10.3916051994283));
#113508=CARTESIAN_POINT('Ctrl Pts',(-22.0438346214652,12.7848480290955,
-10.3362267037117));
#113509=CARTESIAN_POINT('Ctrl Pts',(-22.0387888616031,12.8541212962082,
-10.2786594504841));
#113510=CARTESIAN_POINT('Ctrl Pts',(-22.031539428324,12.9536488087519,-10.1959504090815));
#113511=CARTESIAN_POINT('Ctrl Pts',(-22.0242899950448,13.0494257988114,
-10.1086908709218));
#113512=CARTESIAN_POINT('Ctrl Pts',(-22.0170405617656,13.1410453426988,
-10.0172443800378));
#113513=CARTESIAN_POINT('Ctrl Pts',(-22.0097925827507,13.2326465073522,
-9.92581623367251));
#113514=CARTESIAN_POINT('Ctrl Pts',(-22.0025446037359,13.3200916446911,
-9.8302030543376));
#113515=CARTESIAN_POINT('Ctrl Pts',(-21.995296624721,13.4030103443729,-9.73080556343431));
#113516=CARTESIAN_POINT('Ctrl Pts',(-21.9880484316003,13.485931493478,-9.63140513632318));
#113517=CARTESIAN_POINT('Ctrl Pts',(-21.9808002384797,13.5643257132271,
-9.5282204375736));
#113518=CARTESIAN_POINT('Ctrl Pts',(-21.9735520453591,13.6378623885564,
-9.4216858488588));
#113519=CARTESIAN_POINT('Ctrl Pts',(-21.9663041964995,13.7113955711794,
-9.31515632012281));
#113520=CARTESIAN_POINT('Ctrl Pts',(-21.9590563476398,13.7800714757147,
-9.20527750541117));
#113521=CARTESIAN_POINT('Ctrl Pts',(-21.9518084987802,13.8436025045766,
-9.0925132222994));
#113522=CARTESIAN_POINT('Ctrl Pts',(-21.9445591294989,13.9071468606963,
-8.97972528399588));
#113523=CARTESIAN_POINT('Ctrl Pts',(-21.9373097602177,13.9655440160805,
-8.86405097009453));
#113524=CARTESIAN_POINT('Ctrl Pts',(-21.9300603909364,14.0185518970946,
-8.74597947917628));
#113525=CARTESIAN_POINT('Ctrl Pts',(-21.9275213328559,14.0371176623905,
-8.70462548526845));
#113526=CARTESIAN_POINT('Ctrl Pts',(-21.9249822747754,14.0550227368447,
-8.66297762867487));
#113527=CARTESIAN_POINT('Ctrl Pts',(-21.9224432166949,14.072258099233,-8.62105754707614));
#113528=CARTESIAN_POINT('Ctrl Pts',(-21.9151753922206,14.1215927676882,
-8.50106509895149));
#113529=CARTESIAN_POINT('Ctrl Pts',(-21.9079075677462,14.1654535201482,
-8.37879985409838));
#113530=CARTESIAN_POINT('Ctrl Pts',(-21.9006397432719,14.2036508556539,
-8.25477639656434));
#113531=CARTESIAN_POINT('Ctrl Pts',(-21.8933732460253,14.2418412156796,
-8.13077558781263));
#113532=CARTESIAN_POINT('Ctrl Pts',(-21.8861067487787,14.2743701213767,
-8.0050175340044));
#113533=CARTESIAN_POINT('Ctrl Pts',(-21.8788402515321,14.3010977675838,
-7.87803249683022));
#113534=CARTESIAN_POINT('Ctrl Pts',(-21.8715735448853,14.3278261840071,
-7.75104380030113));
#113535=CARTESIAN_POINT('Ctrl Pts',(-21.8643068382385,14.3487529329938,
-7.6228283840705));
#113536=CARTESIAN_POINT('Ctrl Pts',(-21.8570401315917,14.3637891445478,
-7.49392756590881));
#113537=CARTESIAN_POINT('Ctrl Pts',(-21.8497738247676,14.3788245287919,
-7.36503384002021));
#113538=CARTESIAN_POINT('Ctrl Pts',(-21.8425075179435,14.3879699855593,
-7.23545512785121));
#113539=CARTESIAN_POINT('Ctrl Pts',(-21.8352412111193,14.3911884386049,
-7.10573860345731));
#113540=CARTESIAN_POINT('Ctrl Pts',(-21.8279736222961,14.3944074594842,
-6.97599919309588));
#113541=CARTESIAN_POINT('Ctrl Pts',(-21.8207060334729,14.3916973798453,
-6.84612226427044));
#113542=CARTESIAN_POINT('Ctrl Pts',(-21.8134384446498,14.3830732316722,
-6.71665610505596));
#113543=CARTESIAN_POINT('Ctrl Pts',(-21.8109914870288,14.3801695278977,
-6.67306555354588));
#113544=CARTESIAN_POINT('Ctrl Pts',(-21.8085445294078,14.3765958228007,
-6.62952155223097));
#113545=CARTESIAN_POINT('Ctrl Pts',(-21.8060975717868,14.3723540173125,
-6.58604494473972));
#113546=CARTESIAN_POINT('Ctrl Pts',(-21.7989004737786,14.35987783482,-6.45816965891825));
#113547=CARTESIAN_POINT('Ctrl Pts',(-21.7917033757704,14.3416132490332,
-6.33082772123226));
#113548=CARTESIAN_POINT('Ctrl Pts',(-21.7845062777622,14.3176299764922,
-6.20455276730157));
#113549=CARTESIAN_POINT('Ctrl Pts',(-21.7773108057981,14.2936521225045,
-6.07830634273716));
#113550=CARTESIAN_POINT('Ctrl Pts',(-21.770115333834,14.2639582246201,-5.95312677071234));
#113551=CARTESIAN_POINT('Ctrl Pts',(-21.7629198618699,14.2286692912606,
-5.82953850059646));
#113552=CARTESIAN_POINT('Ctrl Pts',(-21.7557239357197,14.1933781304247,
-5.70594242945247));
#113553=CARTESIAN_POINT('Ctrl Pts',(-21.7485280095695,14.1524913221394,
-5.5839382043744));
#113554=CARTESIAN_POINT('Ctrl Pts',(-21.7413320834193,14.1061801009768,
-5.46403633685718));
#113555=CARTESIAN_POINT('Ctrl Pts',(-21.7341362386062,14.0598694032798,
-5.34413582461646));
#113556=CARTESIAN_POINT('Ctrl Pts',(-21.7269403937931,14.0081345469274,
-5.22633795320274));
#113557=CARTESIAN_POINT('Ctrl Pts',(-21.7197445489799,13.951195264075,-5.11113412108044));
#113558=CARTESIAN_POINT('Ctrl Pts',(-21.7125463803664,13.8942375934544,
-4.9958930854447));
#113559=CARTESIAN_POINT('Ctrl Pts',(-21.7053482117529,13.8320722985288,
-4.8832480808549));
#113560=CARTESIAN_POINT('Ctrl Pts',(-21.6981500431394,13.7649656431987,
-4.77366701566866));
#113561=CARTESIAN_POINT('Ctrl Pts',(-21.6953506710525,13.7388678247307,
-4.73105087375697));
#113562=CARTESIAN_POINT('Ctrl Pts',(-21.6925512989656,13.7120231386475,
-4.68889785170956));
#113563=CARTESIAN_POINT('Ctrl Pts',(-21.6897519268786,13.6844490489701,
-4.64723433822518));
#113564=CARTESIAN_POINT('Ctrl Pts',(-21.6823651612314,13.6116886826953,
-4.53729589467605));
#113565=CARTESIAN_POINT('Ctrl Pts',(-21.6749783955841,13.5338219832499,
-4.43073073882055));
#113566=CARTESIAN_POINT('Ctrl Pts',(-21.6675916299368,13.4511815146991,
-4.32799683478733));
#113567=CARTESIAN_POINT('Ctrl Pts',(-21.6602057767909,13.3685512548839,
-4.2252756216705));
#113568=CARTESIAN_POINT('Ctrl Pts',(-21.652819923645,13.281148602485,-4.12638496293451));
#113569=CARTESIAN_POINT('Ctrl Pts',(-21.645434070499,13.1893468117984,-4.03175026516851));
#113570=CARTESIAN_POINT('Ctrl Pts',(-21.6380488592528,13.0975529995455,
-3.93712379204228));
#113571=CARTESIAN_POINT('Ctrl Pts',(-21.6306636480065,13.0013610322878,
-3.84675277061771));
#113572=CARTESIAN_POINT('Ctrl Pts',(-21.6232784367602,12.9011817562969,
-3.76102651418525));
#113573=CARTESIAN_POINT('Ctrl Pts',(-21.6158945838923,12.8010209065034,
-3.67531602557404));
#113574=CARTESIAN_POINT('Ctrl Pts',(-21.6085107310244,12.6968744537646,
-3.59424880257396));
#113575=CARTESIAN_POINT('Ctrl Pts',(-21.6011268781565,12.5891872591908,
-3.51817467598181));
#113576=CARTESIAN_POINT('Ctrl Pts',(-21.5937442414511,12.4815178013097,
-3.44211307923043));
#113577=CARTESIAN_POINT('Ctrl Pts',(-21.5863616047457,12.3703090248018,
-3.37104312100045));
#113578=CARTESIAN_POINT('Ctrl Pts',(-21.5789789680403,12.2560360828037,
-3.30527223079506));
#113579=CARTESIAN_POINT('Ctrl Pts',(-21.577121406017,12.2272836077984,-3.2887234674252));
#113580=CARTESIAN_POINT('Ctrl Pts',(-21.5752638439937,12.1983372842333,
-3.27250996499309));
#113581=CARTESIAN_POINT('Ctrl Pts',(-21.5734062819704,12.1692049547297,
-3.25663617882909));
#113582=CARTESIAN_POINT('Ctrl Pts',(-21.5663770387532,12.0589646359696,
-3.19656781915905));
#113583=CARTESIAN_POINT('Ctrl Pts',(-21.5593477955361,11.9460238764199,
-3.14134860569491));
#113584=CARTESIAN_POINT('Ctrl Pts',(-21.5523185523189,11.8308409812737,
-3.09121401641908));
#113585=CARTESIAN_POINT('Ctrl Pts',(-21.5452910829351,11.7156871525937,
-3.04109207863409));
#113586=CARTESIAN_POINT('Ctrl Pts',(-21.5382636135512,11.598292668025,-2.99605236218513));
#113587=CARTESIAN_POINT('Ctrl Pts',(-21.5312361441674,11.4791373964743,
-2.95628291073201));
#113588=CARTESIAN_POINT('Ctrl Pts',(-21.5242072492004,11.3599579532428,
-2.91650539170054));
#113589=CARTESIAN_POINT('Ctrl Pts',(-21.5171783542334,11.2390173728664,
-2.88200040031871));
#113590=CARTESIAN_POINT('Ctrl Pts',(-21.5101494592664,11.1168123916017,
-2.85290665147386));
#113591=CARTESIAN_POINT('Ctrl Pts',(-21.5031198947892,10.9945957701737,
-2.82381013141641));
#113592=CARTESIAN_POINT('Ctrl Pts',(-21.496090330312,10.8711148837365,-2.80012596375325));
#113593=CARTESIAN_POINT('Ctrl Pts',(-21.4890607658348,10.7468776224925,
-2.78194193126202));
#113594=CARTESIAN_POINT('Ctrl Pts',(-21.4820266213085,10.6225594155855,
-2.76374605112903));
#113595=CARTESIAN_POINT('Ctrl Pts',(-21.4749924767822,10.4974842312982,
-2.75105751390997));
#113596=CARTESIAN_POINT('Ctrl Pts',(-21.4679583322559,10.3721662707993,
-2.7439123504072));
#113597=CARTESIAN_POINT('Ctrl Pts',(-21.4643257671913,10.3074497095221,
-2.74022245304675));
#113598=CARTESIAN_POINT('Ctrl Pts',(-21.4606932021268,10.2426684536507,
-2.73801005930991));
#113599=CARTESIAN_POINT('Ctrl Pts',(-21.4570606370622,10.1778933606384,
-2.73727468834243));
#113600=CARTESIAN_POINT('Ctrl Pts',(-21.4494486360556,10.0421578502062,
-2.73573372639261));
#113601=CARTESIAN_POINT('Ctrl Pts',(-21.4418366350489,9.90636208137426,
-2.74068047835051));
#113602=CARTESIAN_POINT('Ctrl Pts',(-21.4342246340423,9.77110640803279,
-2.75209192269456));
#113603=CARTESIAN_POINT('Ctrl Pts',(-21.4264321638849,9.63264402511851,
-2.76377391530407));
#113604=CARTESIAN_POINT('Ctrl Pts',(-21.4186396937276,9.49474795528324,
-2.78223096696343));
#113605=CARTESIAN_POINT('Ctrl Pts',(-21.4108472235702,9.35805779034524,
-2.80738197337714));
#113606=CARTESIAN_POINT('Ctrl Pts',(-21.4032412105133,9.22463832793057,
-2.83193117014216));
#113607=CARTESIAN_POINT('Ctrl Pts',(-21.3956351974563,9.09236799004524,
-2.86285756196605));
#113608=CARTESIAN_POINT('Ctrl Pts',(-21.3880291843993,8.96183334801938,
-2.90003370869316));
#113609=CARTESIAN_POINT('Ctrl Pts',(-21.3801434856918,8.82649873181441,
-2.93857688367882));
#113610=CARTESIAN_POINT('Ctrl Pts',(-21.3722577869842,8.69303018501617,
-2.98383817560741));
#113611=CARTESIAN_POINT('Ctrl Pts',(-21.3643720882767,8.56206766416862,
-3.03561797090767));
#113612=CARTESIAN_POINT('Ctrl Pts',(-21.3564863895691,8.43110514332108,
-3.08739776620794));
#113613=CARTESIAN_POINT('Ctrl Pts',(-21.3486006908616,8.30264895994336,
-3.14569598622589));
#113614=CARTESIAN_POINT('Ctrl Pts',(-21.340714992154,8.17732045741597,-3.2102554131556));
#113615=CARTESIAN_POINT('Ctrl Pts',(-21.3336761719785,8.06545151277584,
-3.26788153021242));
#113616=CARTESIAN_POINT('Ctrl Pts',(-21.3266373518029,7.95611455042713,
-3.33047599778825));
#113617=CARTESIAN_POINT('Ctrl Pts',(-21.3195985316273,7.84976015631307,
-3.39778467535514));
#113618=CARTESIAN_POINT('Ctrl Pts',(-21.3125599213837,7.74340893420629,
-3.46509134544864));
#113619=CARTESIAN_POINT('Ctrl Pts',(-21.3055213111402,7.6400404255637,-3.53711173986184));
#113620=CARTESIAN_POINT('Ctrl Pts',(-21.2984827008966,7.54007733081936,
-3.61354769111783));
#113621=CARTESIAN_POINT('Ctrl Pts',(-21.2914403979205,7.44006179149318,
-3.69002374368832));
#113622=CARTESIAN_POINT('Ctrl Pts',(-21.2843980949443,7.34345554026389,
-3.77091974958848));
#113623=CARTESIAN_POINT('Ctrl Pts',(-21.2773557919682,7.25064938419331,
-3.85589629117145));
#113624=CARTESIAN_POINT('Ctrl Pts',(-21.270311531557,7.15781743229572,-3.94089645231006));
#113625=CARTESIAN_POINT('Ctrl Pts',(-21.2632672711458,7.06878795662045,
-4.02997914451082));
#113626=CARTESIAN_POINT('Ctrl Pts',(-21.2562230107345,6.98391525521804,
-4.12276771646865));
#113627=CARTESIAN_POINT('Ctrl Pts',(-21.2491723165041,6.89896503600872,
-4.21564103613083));
#113628=CARTESIAN_POINT('Ctrl Pts',(-21.2421216222736,6.8181794261953,-4.31222670801673));
#113629=CARTESIAN_POINT('Ctrl Pts',(-21.2350709280432,6.74187298426385,
-4.41211433748425));
#113630=CARTESIAN_POINT('Ctrl Pts',(-21.2315037344441,6.70326687792428,
-4.46265099399217));
#113631=CARTESIAN_POINT('Ctrl Pts',(-21.2279365408449,6.6658066369646,-4.51403236253905));
#113632=CARTESIAN_POINT('Ctrl Pts',(-21.2243693472458,6.62952875518707,
-4.56620249702597));
#113633=CARTESIAN_POINT('Ctrl Pts',(-21.2173459196766,6.55810143621733,
-4.66891998366267));
#113634=CARTESIAN_POINT('Ctrl Pts',(-21.2103224921073,6.49113206267362,
-4.77488133278218));
#113635=CARTESIAN_POINT('Ctrl Pts',(-21.203299064538,6.42891752586231,-4.88366865729751));
#113636=CARTESIAN_POINT('Ctrl Pts',(-21.1962814635001,6.3667546013078,-4.99236573346224));
#113637=CARTESIAN_POINT('Ctrl Pts',(-21.1892638624622,6.30933885072374,
-5.10388378270884));
#113638=CARTESIAN_POINT('Ctrl Pts',(-21.1822462614242,6.25692354442136,
-5.21777650231572));
#113639=CARTESIAN_POINT('Ctrl Pts',(-21.1752329179883,6.20454003866059,
-5.33160012282876));
#113640=CARTESIAN_POINT('Ctrl Pts',(-21.1682195745524,6.15715109672532,
-5.44779519409355));
#113641=CARTESIAN_POINT('Ctrl Pts',(-21.1612062311164,6.11496361461179,
-5.5658917019994));
#113642=CARTESIAN_POINT('Ctrl Pts',(-21.1541425572128,6.07247337879379,
-5.6848357161669));
#113643=CARTESIAN_POINT('Ctrl Pts',(-21.1470788833092,6.03525973704695,
-5.80570821283149));
#113644=CARTESIAN_POINT('Ctrl Pts',(-21.1400152094056,6.00348440058743,
-5.92800920087711));
#113645=CARTESIAN_POINT('Ctrl Pts',(-21.133004253243,5.97194621040375,-6.04939742993803));
#113646=CARTESIAN_POINT('Ctrl Pts',(-21.1259932970804,5.94576549596376,
-6.17219251371173));
#113647=CARTESIAN_POINT('Ctrl Pts',(-21.1189823409179,5.925049909777,-6.29589174211361));
#113648=CARTESIAN_POINT('Ctrl Pts',(-21.1119707114441,5.90433233412748,
-6.41960285021839));
#113649=CARTESIAN_POINT('Ctrl Pts',(-21.1049590819704,5.88908099593137,
-6.54421789437491));
#113650=CARTESIAN_POINT('Ctrl Pts',(-21.0979474524966,5.87935206069904,
-6.66922591689215));
#113651=CARTESIAN_POINT('Ctrl Pts',(-21.0909337323132,5.86962022451783,
-6.79427121398003));
#113652=CARTESIAN_POINT('Ctrl Pts',(-21.0839200121298,5.86541410001686,
-6.91970933719594));
#113653=CARTESIAN_POINT('Ctrl Pts',(-21.0769062919464,5.86673779564441,
-7.04502653792429));
#113654=CARTESIAN_POINT('Ctrl Pts',(-21.06980393907,5.8680782188723,-7.17192737767607));
#113655=CARTESIAN_POINT('Ctrl Pts',(-21.0627015861936,5.87508918354248,
-7.29870380973344));
#113656=CARTESIAN_POINT('Ctrl Pts',(-21.0555992333171,5.88772067164072,
-7.42482599909129));
#113657=CARTESIAN_POINT('Ctrl Pts',(-21.0485733140547,5.90021622305687,
-7.54959089532375));
#113658=CARTESIAN_POINT('Ctrl Pts',(-21.0415473947922,5.9182117997394,-7.67371518534136));
#113659=CARTESIAN_POINT('Ctrl Pts',(-21.0345214755298,5.9416072606581,-7.79669530171039));
#113660=CARTESIAN_POINT('Ctrl Pts',(-21.0273809058464,5.96538449360439,
-7.92168223335618));
#113661=CARTESIAN_POINT('Ctrl Pts',(-21.020240336163,5.99473928967706,-8.04548691534146));
#113662=CARTESIAN_POINT('Ctrl Pts',(-21.0130997664796,6.02951374026827,
-8.16759653562821));
#113663=CARTESIAN_POINT('Ctrl Pts',(-21.0059591967962,6.06428819085948,
-8.28970615591497));
#113664=CARTESIAN_POINT('Ctrl Pts',(-20.9988186271128,6.10448211338605,
-8.41012033914232));
#113665=CARTESIAN_POINT('Ctrl Pts',(-20.9916780574294,6.14988677165161,
-8.52834798156522));
#113666=CARTESIAN_POINT('Ctrl Pts',(-20.9848875394138,6.19306556040558,
-8.6407797582169));
#113667=CARTESIAN_POINT('Ctrl Pts',(-20.9780970213983,6.24110041539954,
-8.75160786112374));
#113668=CARTESIAN_POINT('Ctrl Pts',(-20.9713065033827,6.29385322449215,
-8.86037168693147));
#113669=CARTESIAN_POINT('Ctrl Pts',(-20.964525196406,6.34653447672102,-8.96898797939648));
#113670=CARTESIAN_POINT('Ctrl Pts',(-20.9577438894292,6.40392078324138,
-9.07554518694513));
#113671=CARTESIAN_POINT('Ctrl Pts',(-20.9509625824525,6.46582471863268,
-9.17959914495719));
#113672=CARTESIAN_POINT('Ctrl Pts',(-20.9441885968762,6.52766181978393,
-9.28354076169135));
#113673=CARTESIAN_POINT('Ctrl Pts',(-20.9374146112999,6.59400664137681,
-9.38498414360832));
#113674=CARTESIAN_POINT('Ctrl Pts',(-20.9306406257236,6.66462456931131,
-9.48350704645866));
#113675=CARTESIAN_POINT('Ctrl Pts',(-20.923872081502,6.73518577182298,-9.58195080859381));
#113676=CARTESIAN_POINT('Ctrl Pts',(-20.9171035372804,6.81001301240761,
-9.67747841681211));
#113677=CARTESIAN_POINT('Ctrl Pts',(-20.9103349930588,6.88882723169973,
-9.76969475011184));
#113678=CARTESIAN_POINT('Ctrl Pts',(-20.9035692778455,6.96760850947957,
-9.8618725402971));
#113679=CARTESIAN_POINT('Ctrl Pts',(-20.8968035626323,7.05037318437453,
-9.9507414859558));
#113680=CARTESIAN_POINT('Ctrl Pts',(-20.890037847419,7.13680097017415,-10.0359383256054));
#113681=CARTESIAN_POINT('Ctrl Pts',(-20.8832733657405,7.2232129983373,-10.1211196320463));
#113682=CARTESIAN_POINT('Ctrl Pts',(-20.8765088840621,7.31328651177657,
-10.2026298682361));
#113683=CARTESIAN_POINT('Ctrl Pts',(-20.8697444023836,7.40666387645209,
-10.28014213782));
#113684=CARTESIAN_POINT('Ctrl Pts',(-20.8629794634639,7.50004755291707,
-10.3576596468014));
#113685=CARTESIAN_POINT('Ctrl Pts',(-20.8562145245441,7.59673520141363,
-10.4311783842624));
#113686=CARTESIAN_POINT('Ctrl Pts',(-20.8494495856244,7.6963362060632,-10.5004118260392));
#113687=CARTESIAN_POINT('Ctrl Pts',(-20.8426824984199,7.79596884016584,
-10.5696672536977));
#113688=CARTESIAN_POINT('Ctrl Pts',(-20.8359154112155,7.8985163245618,-10.6346344420979));
#113689=CARTESIAN_POINT('Ctrl Pts',(-20.829148324011,8.00355986516484,-10.6950707088088));
#113690=CARTESIAN_POINT('Ctrl Pts',(-20.8223732475449,8.10872742076868,
-10.7555783269196));
#113691=CARTESIAN_POINT('Ctrl Pts',(-20.8155981710788,8.21639654982388,
-10.8115441384382));
#113692=CARTESIAN_POINT('Ctrl Pts',(-20.8088230946128,8.3261246357037,-10.8627718409776));
#113693=CARTESIAN_POINT('Ctrl Pts',(-20.8020434620293,8.43592651175376,
-10.9140339932283));
#113694=CARTESIAN_POINT('Ctrl Pts',(-20.7952638294458,8.54778971316061,
-10.9605515370318));
#113695=CARTESIAN_POINT('Ctrl Pts',(-20.7884841968622,8.66125425324206,
-11.002177335792));
#113696=CARTESIAN_POINT('Ctrl Pts',(-20.7816937465263,8.77489984020051,
-11.0438695537248));
#113697=CARTESIAN_POINT('Ctrl Pts',(-20.7749032961903,8.89015146681934,
-11.0806543242509));
#113698=CARTESIAN_POINT('Ctrl Pts',(-20.7681128458544,9.00653654290877,
-11.1124350540814));
#113699=CARTESIAN_POINT('Ctrl Pts',(-20.7650708197739,9.05867541725731,
-11.1266723732895));
#113700=CARTESIAN_POINT('Ctrl Pts',(-20.7620287936935,9.11104166406988,
-11.1399061162083));
#113701=CARTESIAN_POINT('Ctrl Pts',(-20.7589867676131,9.16359245771118,
-11.1521309733376));
#113702=CARTESIAN_POINT('Ctrl Pts',(-20.7486393029828,9.34234420543419,
-11.1937138767748));
#113703=CARTESIAN_POINT('Ctrl Pts',(-20.7382918383526,9.5237420713755,-11.2237406026673));
#113704=CARTESIAN_POINT('Ctrl Pts',(-20.7279443737223,9.70657007694164,
-11.2419687976436));
#113705=CARTESIAN_POINT('Ctrl Pts',(-20.7200690256185,9.84571857741016,
-11.2558420879492));
#113706=CARTESIAN_POINT('Ctrl Pts',(-20.7121936775147,9.9856955507432,-11.2628818575557));
#113707=CARTESIAN_POINT('Ctrl Pts',(-20.7043183294109,10.1259540174844,
-11.2629985252177));
#113708=CARTESIAN_POINT('Ctrl Pts',(-20.7043183293681,10.1259540182473,
-11.2629985252183));
#113709=CARTESIAN_POINT('Ctrl Pts',(-20.6972124917565,10.2525076480267,
-11.2631037931088));
#113710=CARTESIAN_POINT('Ctrl Pts',(-20.690106654145,10.3792358913459,-11.2575688510535));
#113711=CARTESIAN_POINT('Ctrl Pts',(-20.6830008165335,10.5055936861433,
-11.2463775785066));
#113712=CARTESIAN_POINT('Ctrl Pts',(-20.6761359770942,10.62766599072,-11.235565863779));
#113713=CARTESIAN_POINT('Ctrl Pts',(-20.6692711376549,10.7493921146474,
-11.2194752750085));
#113714=CARTESIAN_POINT('Ctrl Pts',(-20.6624062982156,10.8702797228384,
-11.1981441616781));
#113715=CARTESIAN_POINT('Ctrl Pts',(-20.6555455951751,10.9910944903822,
-11.176825901378));
#113716=CARTESIAN_POINT('Ctrl Pts',(-20.6486848921345,11.1110713460377,
-11.1502734673399));
#113717=CARTESIAN_POINT('Ctrl Pts',(-20.6418241890939,11.2297241573343,
-11.11857691486));
#113718=CARTESIAN_POINT('Ctrl Pts',(-20.6349660822477,11.3483320686035,
-11.0868923568375));
#113719=CARTESIAN_POINT('Ctrl Pts',(-20.6281079754014,11.4656165386136,
-11.0500676597437));
#113720=CARTESIAN_POINT('Ctrl Pts',(-20.6212498685552,11.5811033394191,
-11.0082435985089));
#113721=CARTESIAN_POINT('Ctrl Pts',(-20.6205160050467,11.5934612029986,
-11.0037681429635));
#113722=CARTESIAN_POINT('Ctrl Pts',(-20.6197821415383,11.6057984965267,
-10.9992354896429));
#113723=CARTESIAN_POINT('Ctrl Pts',(-20.6190482780298,11.6181146495903,
-10.9946458447559));
#113724=CARTESIAN_POINT('',(-21.113681670589,10.1291791134783,-11.262999987923));
#113725=CARTESIAN_POINT('Ctrl Pts',(-21.0285562874006,11.6181146495903,
-10.9946458447559));
#113726=CARTESIAN_POINT('Ctrl Pts',(-21.0355840156022,11.5004192767385,
-11.0385053164149));
#113727=CARTESIAN_POINT('Ctrl Pts',(-21.0426117438038,11.3807634475762,
-11.0771668462722));
#113728=CARTESIAN_POINT('Ctrl Pts',(-21.0496394720055,11.2596369012063,
-11.1104695090138));
#113729=CARTESIAN_POINT('Ctrl Pts',(-21.0566691422659,11.1384768824449,
-11.1437813746906));
#113730=CARTESIAN_POINT('Ctrl Pts',(-21.0636988125263,11.015845704538,-11.1717313079601));
#113731=CARTESIAN_POINT('Ctrl Pts',(-21.0707284827866,10.8922472189185,
-11.1942085880452));
#113732=CARTESIAN_POINT('Ctrl Pts',(-21.0773994741671,10.7749551694116,
-11.2155389970329));
#113733=CARTESIAN_POINT('Ctrl Pts',(-21.0840704655475,10.6567923830643,
-11.2319413112385));
#113734=CARTESIAN_POINT('Ctrl Pts',(-21.0907414569279,10.5381962379688,
-11.2433638054108));
#113735=CARTESIAN_POINT('Ctrl Pts',(-21.0983881948149,10.4022533796668,
-11.2564570345833));
#113736=CARTESIAN_POINT('Ctrl Pts',(-21.106034932702,10.2657163342166,-11.2630102654163));
#113737=CARTESIAN_POINT('Ctrl Pts',(-21.113681670589,10.1291791134783,-11.262999987923));
#113738=CARTESIAN_POINT('Ctrl Pts',(-22.5286570444943,11.618114651272,-10.9946458441291));
#113739=CARTESIAN_POINT('Ctrl Pts',(-22.5118635566228,11.897231423232,-10.8906322888935));
#113740=CARTESIAN_POINT('Ctrl Pts',(-22.4949369598826,12.1647784889961,
-10.7576137578564));
#113741=CARTESIAN_POINT('Ctrl Pts',(-22.465868647502,12.6053453742023,-10.4775732694343));
#113742=CARTESIAN_POINT('Ctrl Pts',(-22.4535277673545,12.7845915575229,
-10.342725835719));
#113743=CARTESIAN_POINT('Ctrl Pts',(-22.4257236293028,13.1587098476615,
-10.0121171914199));
#113744=CARTESIAN_POINT('Ctrl Pts',(-22.4102376602721,13.3468564292045,
-9.81026178837383));
#113745=CARTESIAN_POINT('Ctrl Pts',(-22.3707644790326,13.7710499653168,
-9.25626921794873));
#113746=CARTESIAN_POINT('Ctrl Pts',(-22.3475332219828,13.9766060759535,
-8.88452249893456));
#113747=CARTESIAN_POINT('Ctrl Pts',(-22.2991968843045,14.2796126782055,
-8.07143533541486));
#113748=CARTESIAN_POINT('Ctrl Pts',(-22.2738516834091,14.3687709152418,
-7.63244160595406));
#113749=CARTESIAN_POINT('Ctrl Pts',(-22.23441490211,14.399879921126,-6.92636524613201));
#113750=CARTESIAN_POINT('Ctrl Pts',(-22.2200357352687,14.3873239022266,
-6.66458234195366));
#113751=CARTESIAN_POINT('Ctrl Pts',(-22.1818226587369,14.2917628569607,
-5.98591647449479));
#113752=CARTESIAN_POINT('Ctrl Pts',(-22.1576959023024,14.1704129201896,
-5.57739311561262));
#113753=CARTESIAN_POINT('Ctrl Pts',(-22.120506117992,13.8882519171042,-4.97428159231956));
#113754=CARTESIAN_POINT('Ctrl Pts',(-22.1071892271123,13.7672009592946,
-4.76418119343851));
#113755=CARTESIAN_POINT('Ctrl Pts',(-22.0671851319122,13.3567031829939,
-4.17411333030861));
#113756=CARTESIAN_POINT('Ctrl Pts',(-22.0400476309531,13.0207019334589,
-3.83117957033724));
#113757=CARTESIAN_POINT('Ctrl Pts',(-21.9977759452388,12.4066947984301,
-3.38514702377261));
#113758=CARTESIAN_POINT('Ctrl Pts',(-21.9822619869133,12.1625184551894,
-3.24239234048036));
#113759=CARTESIAN_POINT('Ctrl Pts',(-21.9508603667187,11.6519681345354,
-3.0083368422622));
#113760=CARTESIAN_POINT('Ctrl Pts',(-21.935050555265,11.387067969271,-2.91713343544298));
#113761=CARTESIAN_POINT('Ctrl Pts',(-21.8879448747146,10.5757587952574,
-2.72432313185626));
#113762=CARTESIAN_POINT('Ctrl Pts',(-21.8579334985496,10.0164989908293,
-2.70258320307757));
#113763=CARTESIAN_POINT('Ctrl Pts',(-21.8116752950662,9.20696693094667,
-2.82958879436635));
#113764=CARTESIAN_POINT('Ctrl Pts',(-21.7966322572004,8.94955550495293,
-2.89498639316289));
#113765=CARTESIAN_POINT('Ctrl Pts',(-21.7656932431054,8.42658696557584,
-3.08114689744676));
#113766=CARTESIAN_POINT('Ctrl Pts',(-21.749753784929,8.16393679313984,-3.2060725422022));
#113767=CARTESIAN_POINT('Ctrl Pts',(-21.7179039395933,7.67711327384761,
-3.50184230045521));
#113768=CARTESIAN_POINT('Ctrl Pts',(-21.7020905381782,7.45307322008557,
-3.67012909058175));
#113769=CARTESIAN_POINT('Ctrl Pts',(-21.6554089466727,6.84416001296812,
-4.22892638374964));
#113770=CARTESIAN_POINT('Ctrl Pts',(-21.6257875944964,6.5161027709379,-4.67284096003034));
#113771=CARTESIAN_POINT('Ctrl Pts',(-21.5799691432257,6.16697497015337,
-5.40572474724432));
#113772=CARTESIAN_POINT('Ctrl Pts',(-21.5649274230386,6.07559613988268,
-5.65493869451876));
#113773=CARTESIAN_POINT('Ctrl Pts',(-21.5243316192289,5.88959640808551,
-6.35891158709622));
#113774=CARTESIAN_POINT('Ctrl Pts',(-21.4989586169474,5.84505290256321,
-6.82310483597467));
#113775=CARTESIAN_POINT('Ctrl Pts',(-21.4577103596116,5.89390770742929,
-7.55139806143824));
#113776=CARTESIAN_POINT('Ctrl Pts',(-21.4426230694252,5.93668363740592,
-7.8152198623368));
#113777=CARTESIAN_POINT('Ctrl Pts',(-21.4153081095326,6.06029511506826,
-8.29036328542627));
#113778=CARTESIAN_POINT('Ctrl Pts',(-21.4029254648302,6.13379986021384,
-8.50261308988648));
#113779=CARTESIAN_POINT('Ctrl Pts',(-21.3748148471002,6.33555715266349,
-8.96396493236319));
#113780=CARTESIAN_POINT('Ctrl Pts',(-21.359056941832,6.47232512473378,-9.20821749927028));
#113781=CARTESIAN_POINT('Ctrl Pts',(-21.3114335368598,6.95387034171625,
-9.89922444270409));
#113782=CARTESIAN_POINT('Ctrl Pts',(-21.2810313155863,7.36408465176337,
-10.2928121714641));
#113783=CARTESIAN_POINT('Ctrl Pts',(-21.2277055352677,8.16233740054543,
-10.8013827607725));
#113784=CARTESIAN_POINT('Ctrl Pts',(-21.2060291048435,8.51211569060141,
-10.9628682676951));
#113785=CARTESIAN_POINT('Ctrl Pts',(-21.1729824186689,9.08072693148724,
-11.1373756926973));
#113786=CARTESIAN_POINT('Ctrl Pts',(-21.1612647077837,9.28702167925944,
-11.1842599164102));
#113787=CARTESIAN_POINT('Ctrl Pts',(-21.1375559300196,9.70555363933832,
-11.2471601909553));
#113788=CARTESIAN_POINT('Ctrl Pts',(-21.1255964907356,9.91722036984201,
-11.2629838551454));
#113789=CARTESIAN_POINT('Ctrl Pts',(-21.1136182899058,10.1291755310197,
-11.2629999876519));
#113790=CARTESIAN_POINT('Origin',(23.734,10.1295,-7.));
#113791=CARTESIAN_POINT('Ctrl Pts',(18.0286142064722,8.64088528410776,-10.9946458200483));
#113792=CARTESIAN_POINT('Ctrl Pts',(18.039789912646,8.82947631661819,-11.0649247381119));
#113793=CARTESIAN_POINT('Ctrl Pts',(18.0508911903356,9.0228507750007,-11.1217761943531));
#113794=CARTESIAN_POINT('Ctrl Pts',(18.0855389971032,9.6287916599252,-11.2541654000867));
#113795=CARTESIAN_POINT('Ctrl Pts',(18.1093854435775,10.0489723497352,-11.2827744784006));
#113796=CARTESIAN_POINT('Ctrl Pts',(18.1471816832798,10.7245663649431,-11.2291906086153));
#113797=CARTESIAN_POINT('Ctrl Pts',(18.1614166816315,10.9801743034163,-11.1852727903175));
#113798=CARTESIAN_POINT('Ctrl Pts',(18.1906211821946,11.4861716741905,-11.0500376008415));
#113799=CARTESIAN_POINT('Ctrl Pts',(18.2056646969047,11.7351865714645,-10.9579192772123));
#113800=CARTESIAN_POINT('Ctrl Pts',(18.2520848009178,12.4766910552346,-10.60204548056));
#113801=CARTESIAN_POINT('Ctrl Pts',(18.2822647792475,12.9271688953905,-10.2645189885224));
#113802=CARTESIAN_POINT('Ctrl Pts',(18.329563093998,13.4867230231185,-9.64202969247538));
#113803=CARTESIAN_POINT('Ctrl Pts',(18.345361847618,13.6526624310861,-9.41631982831584));
#113804=CARTESIAN_POINT('Ctrl Pts',(18.3745501635932,13.9192880709676,-8.96714577060878));
#113805=CARTESIAN_POINT('Ctrl Pts',(18.3879432541682,14.0251847377267,-8.74808388406812));
#113806=CARTESIAN_POINT('Ctrl Pts',(18.4231081417801,14.2510441149974,-8.15680596322861));
#113807=CARTESIAN_POINT('Ctrl Pts',(18.4452891829018,14.3395625397132,-7.77503814968497));
#113808=CARTESIAN_POINT('Ctrl Pts',(18.4823845661745,14.3994874163579,-7.11696128038773));
#113809=CARTESIAN_POINT('Ctrl Pts',(18.4973478486563,14.3982981455231,-6.84560261077265));
#113810=CARTESIAN_POINT('Ctrl Pts',(18.5347900650453,14.3311933762226,-6.1739546972112));
#113811=CARTESIAN_POINT('Ctrl Pts',(18.5577037585298,14.2339972468066,-5.7794830445814));
#113812=CARTESIAN_POINT('Ctrl Pts',(18.6118397780143,13.8735890188588,-4.88640863501065));
#113813=CARTESIAN_POINT('Ctrl Pts',(18.6422260148492,13.5645771307568,-4.414328195284));
#113814=CARTESIAN_POINT('Ctrl Pts',(18.7055320765152,12.7810685956465,-3.61529310228987));
#113815=CARTESIAN_POINT('Ctrl Pts',(18.7359956167877,12.3137769030668,-3.29648990138105));
#113816=CARTESIAN_POINT('Ctrl Pts',(18.7812358386468,11.5729102061597,-2.98133198485659));
#113817=CARTESIAN_POINT('Ctrl Pts',(18.7951410793747,11.3397496995108,-2.90507356509229));
#113818=CARTESIAN_POINT('Ctrl Pts',(18.8352496442113,10.6462105342338,-2.74269191595506));
#113819=CARTESIAN_POINT('Ctrl Pts',(18.8606370473304,10.1766533737762,-2.71170947289427));
#113820=CARTESIAN_POINT('Ctrl Pts',(18.9017617215762,9.44980269284018,-2.78332847763197));
#113821=CARTESIAN_POINT('Ctrl Pts',(18.9166849818414,9.19107287097638,-2.83326683536358));
#113822=CARTESIAN_POINT('Ctrl Pts',(18.9543381270769,8.54735185340598,-3.02055239473558));
#113823=CARTESIAN_POINT('Ctrl Pts',(18.9765378256604,8.17445315844397,-3.18988433444434));
#113824=CARTESIAN_POINT('Ctrl Pts',(19.0126006065023,7.63363564858332,-3.53605748654641));
#113825=CARTESIAN_POINT('Ctrl Pts',(19.0259264357665,7.4467759557336,-3.67867063866158));
#113826=CARTESIAN_POINT('Ctrl Pts',(19.071107642773,6.85183247790683,-4.21585674879132));
#113827=CARTESIAN_POINT('Ctrl Pts',(19.1018278831666,6.51104879615158,-4.67591755065589));
#113828=CARTESIAN_POINT('Ctrl Pts',(19.1493271776637,6.15427869555142,-5.43625436953596));
#113829=CARTESIAN_POINT('Ctrl Pts',(19.1647097775749,6.06232265312795,-5.69395204102108));
#113830=CARTESIAN_POINT('Ctrl Pts',(19.2024951208292,5.89678902636713,-6.35108753953332));
#113831=CARTESIAN_POINT('Ctrl Pts',(19.2246658134463,5.8543184988969,-6.7555744181102));
#113832=CARTESIAN_POINT('Ctrl Pts',(19.26284741727,5.87964274858108,-7.43003476984898));
#113833=CARTESIAN_POINT('Ctrl Pts',(19.2781161088495,5.91544590216238,-7.698549978111));
#113834=CARTESIAN_POINT('Ctrl Pts',(19.3146038421075,6.06281319314975,-8.33484019050179));
#113835=CARTESIAN_POINT('Ctrl Pts',(19.3355181941132,6.19904208319337,-8.69447252750772));
#113836=CARTESIAN_POINT('Ctrl Pts',(19.3695601003676,6.48666077411959,-9.22523293463471));
#113837=CARTESIAN_POINT('Ctrl Pts',(19.3820628650678,6.60680851926175,-9.41093055469459));
#113838=CARTESIAN_POINT('Ctrl Pts',(19.4101570323969,6.91027278029702,-9.80851650725058));
#113839=CARTESIAN_POINT('Ctrl Pts',(19.4256027430348,7.10115775317109,-10.0133596513102));
#113840=CARTESIAN_POINT('Ctrl Pts',(19.4697929587333,7.6988327593341,-10.5401551096626));
#113841=CARTESIAN_POINT('Ctrl Pts',(19.4992344458114,8.14600379075274,-10.8087494351287));
#113842=CARTESIAN_POINT('Ctrl Pts',(19.5283263127743,8.63383708158961,-10.9920139762997));
#113843=CARTESIAN_POINT('Ctrl Pts',(19.5285362900556,8.63736040044845,-10.9933322634436));
#113844=CARTESIAN_POINT('Ctrl Pts',(19.5287462306467,8.64088535560039,-10.9946458466902));
#113845=CARTESIAN_POINT('',(17.734,10.6581555755053,-11.2300936493755));
#113846=CARTESIAN_POINT('Ctrl Pts',(19.1191572628085,8.64088535679774,-10.9946458471364));
#113847=CARTESIAN_POINT('Ctrl Pts',(19.1119070035151,8.51958773180664,-10.949443987533));
#113848=CARTESIAN_POINT('Ctrl Pts',(19.1046567442216,8.40033276577294,-10.8987066521256));
#113849=CARTESIAN_POINT('Ctrl Pts',(19.0974064849282,8.28362436418113,-10.8426438993342));
#113850=CARTESIAN_POINT('Ctrl Pts',(19.0901561780298,8.16691519628698,-10.7865807784372));
#113851=CARTESIAN_POINT('Ctrl Pts',(19.0829058711315,8.0527529401722,-10.7251923151352));
#113852=CARTESIAN_POINT('Ctrl Pts',(19.0756555642332,7.9416194002362,-10.6587357763546));
#113853=CARTESIAN_POINT('Ctrl Pts',(19.0684059379202,7.83049629239121,-10.5922854758408));
#113854=CARTESIAN_POINT('Ctrl Pts',(19.0611563116072,7.72240162884374,-10.5207682287737));
#113855=CARTESIAN_POINT('Ctrl Pts',(19.0539066852942,7.61779038959773,-10.444486004183));
#113856=CARTESIAN_POINT('Ctrl Pts',(19.0466552587319,7.51315317296975,-10.3681848369578));
#113857=CARTESIAN_POINT('Ctrl Pts',(19.0394038321697,7.41200138947097,-10.2871165304907));
#113858=CARTESIAN_POINT('Ctrl Pts',(19.0321524056074,7.31475933410449,-10.2016252097574));
#113859=CARTESIAN_POINT('Ctrl Pts',(19.0260356350683,7.23273308253644,-10.1295110143619));
#113860=CARTESIAN_POINT('Ctrl Pts',(19.0199188645292,7.15348829353742,-10.0542504741919));
#113861=CARTESIAN_POINT('Ctrl Pts',(19.0138020939901,7.07726035300143,-9.97607159478566));
#113862=CARTESIAN_POINT('Ctrl Pts',(19.0065510835014,6.98689737586705,-9.88339591389356));
#113863=CARTESIAN_POINT('Ctrl Pts',(18.9993000730127,6.90074211026185,-9.78658493399704));
#113864=CARTESIAN_POINT('Ctrl Pts',(18.992049062524,6.81916133806592,-9.68604298984668));
#113865=CARTESIAN_POINT('Ctrl Pts',(18.9847994766285,6.7375965939005,-9.58552079899487));
#113866=CARTESIAN_POINT('Ctrl Pts',(18.9775498907331,6.66060476803244,-9.48126937442019));
#113867=CARTESIAN_POINT('Ctrl Pts',(18.9703003048376,6.58851243587805,-9.37372619961396));
#113868=CARTESIAN_POINT('Ctrl Pts',(18.9630504777803,6.51641770552822,-9.26617944731835));
#113869=CARTESIAN_POINT('Ctrl Pts',(18.9558006507229,6.44922299010419,-9.15534101108407));
#113870=CARTESIAN_POINT('Ctrl Pts',(18.9485508236655,6.38721176553186,-9.04167768517985));
#113871=CARTESIAN_POINT('Ctrl Pts',(18.9413013297149,6.32520339017975,-8.92801958174701));
#113872=CARTESIAN_POINT('Ctrl Pts',(18.9340518357642,6.26837819329272,-8.81153715258735));
#113873=CARTESIAN_POINT('Ctrl Pts',(18.9268023418135,6.21697378950106,-8.6927219654033));
#113874=CARTESIAN_POINT('Ctrl Pts',(18.9195513251248,6.16555858834258,-8.57388182138549));
#113875=CARTESIAN_POINT('Ctrl Pts',(18.912300308436,6.11956659127571,-8.45270825822438));
#113876=CARTESIAN_POINT('Ctrl Pts',(18.9050492917472,6.07918748442404,-8.32971332480681));
#113877=CARTESIAN_POINT('Ctrl Pts',(18.9025183441921,6.06509326755094,-8.28678227949547));
#113878=CARTESIAN_POINT('Ctrl Pts',(18.899987396637,6.05168245386202,-8.24362948664952));
#113879=CARTESIAN_POINT('Ctrl Pts',(18.8974564490819,6.03896168920779,-8.20027718796169));
#113880=CARTESIAN_POINT('Ctrl Pts',(18.8902054210853,6.00251738578437,-8.07607519457316));
#113881=CARTESIAN_POINT('Ctrl Pts',(18.8829543930887,5.97172744130365,-7.95018973388214));
#113882=CARTESIAN_POINT('Ctrl Pts',(18.8757033650922,5.94672659447985,-7.82314982723281));
#113883=CARTESIAN_POINT('Ctrl Pts',(18.868453762145,5.92173066108953,-7.69613488782295));
#113884=CARTESIAN_POINT('Ctrl Pts',(18.8612041591979,5.90252162251066,-7.56796629405867));
#113885=CARTESIAN_POINT('Ctrl Pts',(18.8539545562508,5.88918316891847,-7.43918352888816));
#113886=CARTESIAN_POINT('Ctrl Pts',(18.8467047129841,5.87584427316525,-7.31039649465304));
#113887=CARTESIAN_POINT('Ctrl Pts',(18.8394548697173,5.86837639052481,-7.18099559180068));
#113888=CARTESIAN_POINT('Ctrl Pts',(18.8322050264506,5.86681140365952,-7.05152601894956));
#113889=CARTESIAN_POINT('Ctrl Pts',(18.8249555168243,5.86524648881548,-6.9220624043351));
#113890=CARTESIAN_POINT('Ctrl Pts',(18.817706007198,5.86958392877581,-6.79253047173123));
#113891=CARTESIAN_POINT('Ctrl Pts',(18.8104564975717,5.8798034831745,-6.66347583313945));
#113892=CARTESIAN_POINT('Ctrl Pts',(18.8032054661206,5.89002518287282,-6.53439410326178));
#113893=CARTESIAN_POINT('Ctrl Pts',(18.7959544346696,5.90613143543126,-6.40579021215201));
#113894=CARTESIAN_POINT('Ctrl Pts',(18.7887034032186,5.92805006088456,-6.27820542457924));
#113895=CARTESIAN_POINT('Ctrl Pts',(18.7861725368703,5.93570043613603,-6.23367382275086));
#113896=CARTESIAN_POINT('Ctrl Pts',(18.783641670522,5.94405844734606,-6.1892663079349));
#113897=CARTESIAN_POINT('Ctrl Pts',(18.7811108041737,5.95311955176749,-6.14500564234539));
#113898=CARTESIAN_POINT('Ctrl Pts',(18.773859872354,5.97907961497491,-6.0181988401207));
#113899=CARTESIAN_POINT('Ctrl Pts',(18.7666089405343,6.01082393879235,-5.89255237034654));
#113900=CARTESIAN_POINT('Ctrl Pts',(18.7593580087146,6.04822384784453,-5.76859674767075));
#113901=CARTESIAN_POINT('Ctrl Pts',(18.7521085017796,6.08561640741904,-5.64466548358579));
#113902=CARTESIAN_POINT('Ctrl Pts',(18.7448589948447,6.12866223542571,-5.52242473459185));
#113903=CARTESIAN_POINT('Ctrl Pts',(18.7376094879098,6.17718265209152,-5.4023903538656));
#113904=CARTESIAN_POINT('Ctrl Pts',(18.7303597394478,6.22570468528001,-5.28235197403316));
#113905=CARTESIAN_POINT('Ctrl Pts',(18.7231099909859,6.27970154543043,-5.16452043124017));
#113906=CARTESIAN_POINT('Ctrl Pts',(18.7158602425239,6.33894610020495,-5.04939236832506));
#113907=CARTESIAN_POINT('Ctrl Pts',(18.7086108267425,6.39818793633194,-4.93426958847141));
#113908=CARTESIAN_POINT('Ctrl Pts',(18.7013614109611,6.46267682563546,-4.82185034692949));
#113909=CARTESIAN_POINT('Ctrl Pts',(18.6941119951796,6.53213938755326,-4.71260724316597));
#113910=CARTESIAN_POINT('Ctrl Pts',(18.6868610553831,6.60161655230259,-4.6033411736696));
#113911=CARTESIAN_POINT('Ctrl Pts',(18.6796101155865,6.67606929206711,-4.49725286707198));
#113912=CARTESIAN_POINT('Ctrl Pts',(18.6723591757899,6.75518036948062,-4.39478675899811));
#113913=CARTESIAN_POINT('Ctrl Pts',(18.6698278369485,6.78279843674699,-4.3590153353514));
#113914=CARTESIAN_POINT('Ctrl Pts',(18.667296498107,6.81098385947148,-4.32368509049485));
#113915=CARTESIAN_POINT('Ctrl Pts',(18.6647651592655,6.83972195599233,-4.28881401944369));
#113916=CARTESIAN_POINT('Ctrl Pts',(18.6575139800672,6.92204403957849,-4.18892364487664));
#113917=CARTESIAN_POINT('Ctrl Pts',(18.6502628008689,7.00893389101168,-4.09276746335985));
#113918=CARTESIAN_POINT('Ctrl Pts',(18.6430116216706,7.1000293559808,-4.00075399191298));
#113919=CARTESIAN_POINT('Ctrl Pts',(18.6357618670361,7.19110692437069,-3.90875859739654));
#113920=CARTESIAN_POINT('Ctrl Pts',(18.6285121124016,7.28638821505115,-3.82090453494306));
#113921=CARTESIAN_POINT('Ctrl Pts',(18.6212623577671,7.38547375701612,-3.7375639503868));
#113922=CARTESIAN_POINT('Ctrl Pts',(18.6140123636244,7.48456257244293,-3.65422061253054));
#113923=CARTESIAN_POINT('Ctrl Pts',(18.6067623694818,7.58745562811984,-3.57539127582746));
#113924=CARTESIAN_POINT('Ctrl Pts',(18.5995123753391,7.69371963756569,-3.50140842252495));
#113925=CARTESIAN_POINT('Ctrl Pts',(18.5922627157194,7.79997874386997,-3.42742898287495));
#113926=CARTESIAN_POINT('Ctrl Pts',(18.5850130560997,7.9096082081335,-3.35829577537722));
#113927=CARTESIAN_POINT('Ctrl Pts',(18.5777633964799,8.02214513874008,-3.29429838104521));
#113928=CARTESIAN_POINT('Ctrl Pts',(18.5705122175814,8.13470565320906,-3.23028757506482));
#113929=CARTESIAN_POINT('Ctrl Pts',(18.5632610386828,8.25017455020292,-3.17141490238704));
#113930=CARTESIAN_POINT('Ctrl Pts',(18.5560098597843,8.36806337543537,-3.11792452190296));
#113931=CARTESIAN_POINT('Ctrl Pts',(18.553479744642,8.4091976938689,-3.09926040900147));
#113932=CARTESIAN_POINT('Ctrl Pts',(18.5509496294997,8.45062643100319,-3.08125116393092));
#113933=CARTESIAN_POINT('Ctrl Pts',(18.5484195143573,8.49232821961963,-3.06390579869763));
#113934=CARTESIAN_POINT('Ctrl Pts',(18.5411687396156,8.61183672361191,-3.01419765142135));
#113935=CARTESIAN_POINT('Ctrl Pts',(18.5339179648738,8.73363233864965,-2.96992735561749));
#113936=CARTESIAN_POINT('Ctrl Pts',(18.526667190132,8.85720382874785,-2.93128626558502));
#113937=CARTESIAN_POINT('Ctrl Pts',(18.5194178403275,8.98075103432083,-2.89265276937961));
#113938=CARTESIAN_POINT('Ctrl Pts',(18.512168490523,9.10607308895427,-2.85964637530119));
#113939=CARTESIAN_POINT('Ctrl Pts',(18.5049191407185,9.23264281572258,-2.83240882631106));
#113940=CARTESIAN_POINT('Ctrl Pts',(18.4976695478915,9.35921678553134,-2.80517036422721));
#113941=CARTESIAN_POINT('Ctrl Pts',(18.4904199550646,9.48703817382436,-2.7837012099904));
#113942=CARTESIAN_POINT('Ctrl Pts',(18.4831703622376,9.61556849839147,-2.76809222552589));
#113943=CARTESIAN_POINT('Ctrl Pts',(18.4759211008008,9.7440929476379,-2.7524839545723));
#113944=CARTESIAN_POINT('Ctrl Pts',(18.468671839364,9.8733259249023,-2.74273535747441));
#113945=CARTESIAN_POINT('Ctrl Pts',(18.4614225779272,10.0027228802262,-2.7388855258393));
#113946=CARTESIAN_POINT('Ctrl Pts',(18.4541717893004,10.1321470953937,-2.73503488316649));
#113947=CARTESIAN_POINT('Ctrl Pts',(18.4469210006736,10.2617350119484,-2.73708549773513));
#113948=CARTESIAN_POINT('Ctrl Pts',(18.4396702120468,10.3909407646312,-2.74502435652223));
#113949=CARTESIAN_POINT('Ctrl Pts',(18.4371380978476,10.4360618870127,-2.74779675799403));
#113950=CARTESIAN_POINT('Ctrl Pts',(18.4346059836484,10.4811364186229,-2.7512867892791));
#113951=CARTESIAN_POINT('Ctrl Pts',(18.4320738694491,10.5261412037448,-2.75549240129178));
#113952=CARTESIAN_POINT('Ctrl Pts',(18.4248227506678,10.6550196890614,-2.76753585188386));
#113953=CARTESIAN_POINT('Ctrl Pts',(18.4175716318865,10.7833724865782,-2.78545561878685));
#113954=CARTESIAN_POINT('Ctrl Pts',(18.4103205131052,10.9106582237015,-2.80918136522904));
#113955=CARTESIAN_POINT('Ctrl Pts',(18.4030708203354,11.0379189286979,-2.83290244574471));
#113956=CARTESIAN_POINT('Ctrl Pts',(18.3958211275656,11.1641126522594,-2.86242716480153));
#113957=CARTESIAN_POINT('Ctrl Pts',(18.3885714347958,11.2887071690741,-2.89763388528435));
#113958=CARTESIAN_POINT('Ctrl Pts',(18.3813215040001,11.4133057766442,-2.93284176169347));
#113959=CARTESIAN_POINT('Ctrl Pts',(18.3740715732044,11.536304738905,-2.97373192183976));
#113960=CARTESIAN_POINT('Ctrl Pts',(18.3668216424088,11.6571856682521,-3.02013247720264));
#113961=CARTESIAN_POINT('Ctrl Pts',(18.3595720468175,11.7780610086043,-3.06653088721086));
#113962=CARTESIAN_POINT('Ctrl Pts',(18.3523224512263,11.8968181898397,-3.11843905729658));
#113963=CARTESIAN_POINT('Ctrl Pts',(18.3450728556351,12.0129577051053,-3.17563651399614));
#113964=CARTESIAN_POINT('Ctrl Pts',(18.3378217412121,12.1291215522637,-3.2328459538901));
#113965=CARTESIAN_POINT('Ctrl Pts',(18.3305706267891,12.2426663281592,-3.29534674046882));
#113966=CARTESIAN_POINT('Ctrl Pts',(18.3233195123661,12.3531157624676,-3.3628717453318));
#113967=CARTESIAN_POINT('Ctrl Pts',(18.3207890830911,12.3916594215088,-3.38643601961256));
#113968=CARTESIAN_POINT('Ctrl Pts',(18.318258653816,12.4298263586739,-3.41061174409129));
#113969=CARTESIAN_POINT('Ctrl Pts',(18.3157282245409,12.4675971128062,-3.43538629146338));
#113970=CARTESIAN_POINT('Ctrl Pts',(18.308476572844,12.5758397560588,-3.50638467512143));
#113971=CARTESIAN_POINT('Ctrl Pts',(18.3012249211471,12.6808655344705,-3.58232974729542));
#113972=CARTESIAN_POINT('Ctrl Pts',(18.2939732694502,12.7822289939055,-3.66290577224841));
#113973=CARTESIAN_POINT('Ctrl Pts',(18.2867230375805,12.8835726070214,-3.74346602092941));
#113974=CARTESIAN_POINT('Ctrl Pts',(18.2794728057108,12.9812550611857,-3.82865519873923));
#113975=CARTESIAN_POINT('Ctrl Pts',(18.272222573841,13.0748630102606,-3.91811652754548));
#113976=CARTESIAN_POINT('Ctrl Pts',(18.2649721003639,13.1684740787353,-4.00758083756907));
#113977=CARTESIAN_POINT('Ctrl Pts',(18.2577216268868,13.2580101184567,-4.10131734695304));
#113978=CARTESIAN_POINT('Ctrl Pts',(18.2504711534097,13.3430935434766,-4.19893135797681));
#113979=CARTESIAN_POINT('Ctrl Pts',(18.2432210145619,13.428173041662,-4.29654086384509));
#113980=CARTESIAN_POINT('Ctrl Pts',(18.2359708757141,13.5088001104695,-4.39802725173114));
#113981=CARTESIAN_POINT('Ctrl Pts',(18.2287207368664,13.584636598925,-4.50296173782437));
#113982=CARTESIAN_POINT('Ctrl Pts',(18.2214690829431,13.6604889350776,-4.60791815227929));
#113983=CARTESIAN_POINT('Ctrl Pts',(18.2142174290198,13.7315484893428,-4.71632382367757));
#113984=CARTESIAN_POINT('Ctrl Pts',(18.2069657750966,13.7975194901171,-4.82771962672384));
#113985=CARTESIAN_POINT('Ctrl Pts',(18.2044380432753,13.8205152093976,-4.86654921223581));
#113986=CARTESIAN_POINT('Ctrl Pts',(18.201910311454,13.8428930454219,-4.90574186097849));
#113987=CARTESIAN_POINT('Ctrl Pts',(18.1993825796327,13.8646417522872,-4.94527736900554));
#113988=CARTESIAN_POINT('Ctrl Pts',(18.192134450428,13.927004949233,-5.05864322053447));
#113989=CARTESIAN_POINT('Ctrl Pts',(18.1848863212232,13.9842146238742,-5.17487118894443));
#113990=CARTESIAN_POINT('Ctrl Pts',(18.1776381920185,14.0360251498106,-5.29347421528507));
#113991=CARTESIAN_POINT('Ctrl Pts',(18.1703915005286,14.0878253987829,-5.41205371592257));
#113992=CARTESIAN_POINT('Ctrl Pts',(18.1631448090387,14.1342284968229,-5.53300701759747));
#113993=CARTESIAN_POINT('Ctrl Pts',(18.1558981175488,14.1750364017306,-5.65582582145293));
#113994=CARTESIAN_POINT('Ctrl Pts',(18.1486511750523,14.2158457201186,-5.77864887943421));
#113995=CARTESIAN_POINT('Ctrl Pts',(18.1414042325558,14.2510593454277,-5.90333724128653));
#113996=CARTESIAN_POINT('Ctrl Pts',(18.1341572900592,14.2805285869955,-6.02936584134581));
#113997=CARTESIAN_POINT('Ctrl Pts',(18.1269106671075,14.309996529154,-6.15538888433221));
#113998=CARTESIAN_POINT('Ctrl Pts',(18.1196640441559,14.3337205171969,-6.28275170972903));
#113999=CARTESIAN_POINT('Ctrl Pts',(18.1124174212041,14.3516026666731,-6.41091760162758));
#114000=CARTESIAN_POINT('Ctrl Pts',(18.1051692316137,14.3694886820697,-6.53911120155683));
#114001=CARTESIAN_POINT('Ctrl Pts',(18.0979210420233,14.3815302891234,-6.66810787166596));
#114002=CARTESIAN_POINT('Ctrl Pts',(18.0906728524328,14.3876812579306,-6.79736393556808));
#114003=CARTESIAN_POINT('Ctrl Pts',(18.0881275465301,14.3898412589926,-6.84275405931048));
#114004=CARTESIAN_POINT('Ctrl Pts',(18.0855822406273,14.3912753162859,-6.88817613537974));
#114005=CARTESIAN_POINT('Ctrl Pts',(18.0830369347245,14.3919829512416,-6.93360654870618));
#114006=CARTESIAN_POINT('Ctrl Pts',(18.0757781803886,14.3940009987767,-7.06316591104304));
#114007=CARTESIAN_POINT('Ctrl Pts',(18.0685194260528,14.3901080601192,-7.19283957595163));
#114008=CARTESIAN_POINT('Ctrl Pts',(18.0612606717169,14.3803155764213,-7.32208063470887));
#114009=CARTESIAN_POINT('Ctrl Pts',(18.0540033125099,14.3705249748337,-7.45129685340011));
#114010=CARTESIAN_POINT('Ctrl Pts',(18.0467459533029,14.3548371161971,-7.58008028877821));
#114011=CARTESIAN_POINT('Ctrl Pts',(18.0394885940959,14.3333154303526,-7.70788758113798));
#114012=CARTESIAN_POINT('Ctrl Pts',(18.0322310294306,14.3117931352219,-7.83569849176514));
#114013=CARTESIAN_POINT('Ctrl Pts',(18.0249734647654,14.2844367364672,-7.96253286415625));
#114014=CARTESIAN_POINT('Ctrl Pts',(18.0177159001001,14.2513611175704,-8.08785565561839));
#114015=CARTESIAN_POINT('Ctrl Pts',(18.0104587108012,14.2182872093681,-8.21317196529727));
#114016=CARTESIAN_POINT('Ctrl Pts',(18.0032015215023,14.1794947619858,-8.33697651802529));
#114017=CARTESIAN_POINT('Ctrl Pts',(17.9959443322034,14.1351490069288,-8.45874776205162));
#114018=CARTESIAN_POINT('Ctrl Pts',(17.9886857467642,14.0907947206216,-8.58054243246768));
#114019=CARTESIAN_POINT('Ctrl Pts',(17.981427161325,14.0408851109871,-8.7003026895735));
#114020=CARTESIAN_POINT('Ctrl Pts',(17.9741685758858,13.9856343135614,-8.817525008294));
#114021=CARTESIAN_POINT('Ctrl Pts',(17.971676147196,13.9666624803039,-8.85777641439939));
#114022=CARTESIAN_POINT('Ctrl Pts',(17.9691837185061,13.9470612951703,-8.8977287593196));
#114023=CARTESIAN_POINT('Ctrl Pts',(17.9666912898163,13.9268407111584,-8.93736225920162));
#114024=CARTESIAN_POINT('Ctrl Pts',(17.959457012044,13.868150437668,-9.05239854826719));
#114025=CARTESIAN_POINT('Ctrl Pts',(17.9522227342717,13.8042175019266,-9.16478836006122));
#114026=CARTESIAN_POINT('Ctrl Pts',(17.9449884564993,13.735305827901,-9.2740565805352));
#114027=CARTESIAN_POINT('Ctrl Pts',(17.9377556208397,13.6664078910309,-9.38330301900235));
#114028=CARTESIAN_POINT('Ctrl Pts',(17.9305227851801,13.5925333815593,-9.48942881237161));
#114029=CARTESIAN_POINT('Ctrl Pts',(17.9232899495204,13.5139905279122,-9.5919862782184));
#114030=CARTESIAN_POINT('Ctrl Pts',(17.9160567323261,13.435443531101,-9.69454915400889));
#114031=CARTESIAN_POINT('Ctrl Pts',(17.9088235151317,13.3522279072543,-9.79354304685971));
#114032=CARTESIAN_POINT('Ctrl Pts',(17.9015902979374,13.2646934763842,-9.88855168997165));
#114033=CARTESIAN_POINT('Ctrl Pts',(17.8943572886278,13.1771615612799,-9.98355760250672));
#114034=CARTESIAN_POINT('Ctrl Pts',(17.8871242793183,13.0853113257864,-10.0745782395425));
#114035=CARTESIAN_POINT('Ctrl Pts',(17.8798912700088,12.9895307352709,-10.1612328597093));
#114036=CARTESIAN_POINT('Ctrl Pts',(17.8726564173338,12.8937257346344,-10.2479095642018));
#114037=CARTESIAN_POINT('Ctrl Pts',(17.8654215646588,12.7939886377373,-10.3302177959126));
#114038=CARTESIAN_POINT('Ctrl Pts',(17.8581867119838,12.6907421457889,-10.4078156743924));
#114039=CARTESIAN_POINT('Ctrl Pts',(17.8555730229586,12.6534429449591,-10.4358489644226));
#114040=CARTESIAN_POINT('Ctrl Pts',(17.8529593339334,12.6156860341656,-10.4632678865055));
#114041=CARTESIAN_POINT('Ctrl Pts',(17.8503456449081,12.5774923427427,-10.4900576628293));
#114042=CARTESIAN_POINT('Ctrl Pts',(17.843054929369,12.4709535246718,-10.5647860014525));
#114043=CARTESIAN_POINT('Ctrl Pts',(17.83576421383,12.3609735972743,-10.6346442279424));
#114044=CARTESIAN_POINT('Ctrl Pts',(17.8284734982909,12.2480155917303,-10.6993324651342));
#114045=CARTESIAN_POINT('Ctrl Pts',(17.8211843011505,12.1350811113517,-10.7640072300494));
#114046=CARTESIAN_POINT('Ctrl Pts',(17.8138951040101,12.0191700832606,-10.8235139860041));
#114047=CARTESIAN_POINT('Ctrl Pts',(17.8066059068697,11.9007717818896,-10.8775978742878));
#114048=CARTESIAN_POINT('Ctrl Pts',(17.7993170289403,11.7823786654573,-10.9316793941115));
#114049=CARTESIAN_POINT('Ctrl Pts',(17.7920281510109,11.661498799066,-10.9803383769681));
#114050=CARTESIAN_POINT('Ctrl Pts',(17.7847392730815,11.5386434575797,-11.0233672111753));
#114051=CARTESIAN_POINT('Ctrl Pts',(17.7774511732815,11.4158012316036,-11.0663914518083));
#114052=CARTESIAN_POINT('Ctrl Pts',(17.7701630734815,11.2909842708733,-11.1037866334837));
#114053=CARTESIAN_POINT('Ctrl Pts',(17.7628749736815,11.1647210635762,-11.1353943402689));
#114054=CARTESIAN_POINT('Ctrl Pts',(17.755586336441,11.0384485453526,-11.167004377876));
#114055=CARTESIAN_POINT('Ctrl Pts',(17.7482976992005,10.910729895161,-11.1928260056546));
#114056=CARTESIAN_POINT('Ctrl Pts',(17.74100906196,10.7821062475066,-11.2127513676593));
#114057=CARTESIAN_POINT('Ctrl Pts',(17.7386727079734,10.740876266913,-11.2191383913813));
#114058=CARTESIAN_POINT('Ctrl Pts',(17.7363363539867,10.6995533730216,-11.2249199633334));
#114059=CARTESIAN_POINT('Ctrl Pts',(17.734,10.6581555755053,-11.2300936493755));
#114060=CARTESIAN_POINT('Origin',(17.734,10.1295,-7.));
#114061=CARTESIAN_POINT('Origin',(-18.734,-18.952,1.76670989022851));
#114062=CARTESIAN_POINT('',(-21.2964370736898,-18.9538544369521,-1.0332901097715));
#114063=CARTESIAN_POINT('Ctrl Pts',(-17.1722616763361,-16.9190322283098,
-0.516748667021866));
#114064=CARTESIAN_POINT('Ctrl Pts',(-16.5519397059328,-17.4014734539573,
-0.555987270520924));
#114065=CARTESIAN_POINT('Ctrl Pts',(-15.7420434198304,-19.0426368321606,
-0.637617809580458));
#114066=CARTESIAN_POINT('Ctrl Pts',(-17.1190396890662,-21.5123500683105,
-0.76164028420047));
#114067=CARTESIAN_POINT('Ctrl Pts',(-20.0126665309401,-21.6957542121544,
-0.888816090881905));
#114068=CARTESIAN_POINT('Ctrl Pts',(-21.2376962809792,-20.0341121664399,
-0.979366032738912));
#114069=CARTESIAN_POINT('Ctrl Pts',(-21.2973788721029,-19.0694704700222,
-1.02752403903544));
#114070=CARTESIAN_POINT('Ctrl Pts',(-21.2964370736898,-18.9538544369521,
-1.0332901097715));
#114071=CARTESIAN_POINT('Ctrl Pts',(-21.2964370736898,-18.9538544369521,
-1.0332901097715));
#114072=CARTESIAN_POINT('Ctrl Pts',(-21.2904548055299,-18.219465735772,
-1.06991597459592));
#114073=CARTESIAN_POINT('Ctrl Pts',(-20.5735369171316,-16.6248681111266,
-1.14893377498083));
#114074=CARTESIAN_POINT('Ctrl Pts',(-18.4657781175424,-16.1791426091993,
-1.24342933697954));
#114075=CARTESIAN_POINT('Ctrl Pts',(-17.4224626768032,-16.7324608551944,
-1.30129903415381));
#114076=CARTESIAN_POINT('Ctrl Pts',(-17.1763037562512,-16.9242236971175,
-1.31677679576762));
#114077=CARTESIAN_POINT('',(-21.2938947462506,-18.950658323174,-0.966709917955182));
#114078=CARTESIAN_POINT('Ctrl Pts',(-21.2939996483808,-18.9506582509922,
-0.966709918807928));
#114079=CARTESIAN_POINT('Ctrl Pts',(-21.2939507847444,-18.8574285254183,
-0.971325634427595));
#114080=CARTESIAN_POINT('Ctrl Pts',(-21.2888049399727,-18.7643768813754,
-0.975941350047264));
#114081=CARTESIAN_POINT('Ctrl Pts',(-21.2786450004472,-18.6720324631339,
-0.980557065666932));
#114082=CARTESIAN_POINT('Ctrl Pts',(-21.2684492555577,-18.5793626073736,
-0.98518904785764));
#114083=CARTESIAN_POINT('Ctrl Pts',(-21.2532041411694,-18.4874052362913,
-0.989821030048348));
#114084=CARTESIAN_POINT('Ctrl Pts',(-21.2330434185021,-18.3966784783199,
-0.994453012239056));
#114085=CARTESIAN_POINT('Ctrl Pts',(-21.2127838652416,-18.3055069654919,
-0.999107701033865));
#114086=CARTESIAN_POINT('Ctrl Pts',(-21.1875605220101,-18.2155784195034,
-1.00376238982867));
#114087=CARTESIAN_POINT('Ctrl Pts',(-21.1575575881288,-18.1273979038206,
-1.00841707862348));
#114088=CARTESIAN_POINT('Ctrl Pts',(-21.1382431842027,-18.0706316520587,
-1.01141353689948));
#114089=CARTESIAN_POINT('Ctrl Pts',(-21.1169490236919,-18.0145893782908,
-1.01440999517548));
#114090=CARTESIAN_POINT('Ctrl Pts',(-21.0937343882856,-17.9594005758905,
-1.01740645345148));
#114091=CARTESIAN_POINT('Ctrl Pts',(-21.0613129620801,-17.8823242120765,
-1.02159128983477));
#114092=CARTESIAN_POINT('Ctrl Pts',(-21.0250509387666,-17.8066946664276,
-1.02577612621805));
#114093=CARTESIAN_POINT('Ctrl Pts',(-20.9850989461096,-17.7329210301116,
-1.02996096260134));
#114094=CARTESIAN_POINT('Ctrl Pts',(-20.9452038038474,-17.6592523712966,
-1.03413984409765));
#114095=CARTESIAN_POINT('Ctrl Pts',(-20.9016293390032,-17.5874347771646,
-1.03831872559397));
#114096=CARTESIAN_POINT('Ctrl Pts',(-20.8545742066751,-17.5178573871528,
-1.04249760709029));
#114097=CARTESIAN_POINT('Ctrl Pts',(-20.8066785470568,-17.447037163635,
-1.0467511343004));
#114098=CARTESIAN_POINT('Ctrl Pts',(-20.7551768351364,-17.378538408205,
-1.05100466151051));
#114099=CARTESIAN_POINT('Ctrl Pts',(-20.700327539557,-17.3127452891086,
-1.05525818872062));
#114100=CARTESIAN_POINT('Ctrl Pts',(-20.6465383152431,-17.2482237523413,
-1.05942950809333));
#114101=CARTESIAN_POINT('Ctrl Pts',(-20.5895300617654,-17.1863045680918,
-1.06360082746604));
#114102=CARTESIAN_POINT('Ctrl Pts',(-20.5295891698328,-17.1273193339164,
-1.06777214683875));
#114103=CARTESIAN_POINT('Ctrl Pts',(-20.4696683865407,-17.0683538877827,
-1.0719420668402));
#114104=CARTESIAN_POINT('Ctrl Pts',(-20.4068172462802,-17.0123207593135,
-1.07611198684164));
#114105=CARTESIAN_POINT('Ctrl Pts',(-20.3413596900249,-16.9595154136398,
-1.08028190684309));
#114106=CARTESIAN_POINT('Ctrl Pts',(-20.2759044627329,-16.9067119467669,
-1.08445167847984));
#114107=CARTESIAN_POINT('Ctrl Pts',(-20.2078433623746,-16.8571363224976,
-1.08862145011659));
#114108=CARTESIAN_POINT('Ctrl Pts',(-20.1375330967625,-16.8110434739836,
-1.09279122175334));
#114109=CARTESIAN_POINT('Ctrl Pts',(-20.0647584945777,-16.763335096196,
-1.0971071416183));
#114110=CARTESIAN_POINT('Ctrl Pts',(-19.9895745735351,-16.719358459641,
-1.10142306148326));
#114111=CARTESIAN_POINT('Ctrl Pts',(-19.912407443714,-16.6793460675678,
-1.10573898134823));
#114112=CARTESIAN_POINT('Ctrl Pts',(-19.8377461836544,-16.6406330090789,
-1.10991474914186));
#114113=CARTESIAN_POINT('Ctrl Pts',(-19.7612289942278,-16.6056308240551,
-1.1140905169355));
#114114=CARTESIAN_POINT('Ctrl Pts',(-19.6832631274215,-16.5745014164215,
-1.11826628472913));
#114115=CARTESIAN_POINT('Ctrl Pts',(-19.6013720862764,-16.5418048056381,
-1.12265228062976));
#114116=CARTESIAN_POINT('Ctrl Pts',(-19.5178832247938,-16.513381343314,
-1.12703827653039));
#114117=CARTESIAN_POINT('Ctrl Pts',(-19.4332853705762,-16.4893591470744,
-1.13142427243102));
#114118=CARTESIAN_POINT('Ctrl Pts',(-19.3486875163586,-16.4653369508349,
-1.13581026833165));
#114119=CARTESIAN_POINT('Ctrl Pts',(-19.262981251447,-16.4457160760172,
-1.14019626423228));
#114120=CARTESIAN_POINT('Ctrl Pts',(-19.1766642016327,-16.4305622346382,
-1.14458226013291));
#114121=CARTESIAN_POINT('Ctrl Pts',(-19.090189137421,-16.4153806522147,
-1.14897628515989));
#114122=CARTESIAN_POINT('Ctrl Pts',(-19.0027632421913,-16.4046231875652,
-1.15337031018687));
#114123=CARTESIAN_POINT('Ctrl Pts',(-18.9148794933972,-16.3983981107329,
-1.15776433521386));
#114124=CARTESIAN_POINT('Ctrl Pts',(-18.8313212938358,-16.3924794258865,
-1.161942090773));
#114125=CARTESIAN_POINT('Ctrl Pts',(-18.7473497761972,-16.3906576251858,
-1.16611984633214));
#114126=CARTESIAN_POINT('Ctrl Pts',(-18.6633997116546,-16.3929737009391,
-1.17029760189128));
#114127=CARTESIAN_POINT('Ctrl Pts',(-18.579531146622,-16.3952875282243,
-1.17447130164614));
#114128=CARTESIAN_POINT('Ctrl Pts',(-18.4956844505271,-16.4017312432599,
-1.178645001401));
#114129=CARTESIAN_POINT('Ctrl Pts',(-18.4122970204125,-16.4122938766612,
-1.18281870115586));
#114130=CARTESIAN_POINT('Ctrl Pts',(-18.3289655293808,-16.4228494242941,
-1.18698960105303));
#114131=CARTESIAN_POINT('Ctrl Pts',(-18.2460931473904,-16.4375183441828,
-1.19116050095021));
#114132=CARTESIAN_POINT('Ctrl Pts',(-18.1641134026781,-16.4562377384469,
-1.19533140084739));
#114133=CARTESIAN_POINT('Ctrl Pts',(-18.0821640628827,-16.4749501900005,
-1.19950075382751));
#114134=CARTESIAN_POINT('Ctrl Pts',(-18.0011071501552,-16.4977100272984,
-1.20367010680763));
#114135=CARTESIAN_POINT('Ctrl Pts',(-17.9213658855002,-16.5244032880334,
-1.20783945978775));
#114136=CARTESIAN_POINT('Ctrl Pts',(-17.8416024611271,-16.5511039666986,
-1.21200997141123));
#114137=CARTESIAN_POINT('Ctrl Pts',(-17.7631558535378,-16.5817401119467,
-1.21618048303471));
#114138=CARTESIAN_POINT('Ctrl Pts',(-17.686433123936,-16.6161481981569,
-1.22035099465819));
#114139=CARTESIAN_POINT('Ctrl Pts',(-17.6096979315643,-16.6505618735851,
-1.22452218373576));
#114140=CARTESIAN_POINT('Ctrl Pts',(-17.5346875892803,-16.6887485101164,
-1.22869337281333));
#114141=CARTESIAN_POINT('Ctrl Pts',(-17.4617864601774,-16.7304976459405,
-1.2328645618909));
#114142=CARTESIAN_POINT('Ctrl Pts',(-17.3888184724273,-16.7722850704821,
-1.23703957642442));
#114143=CARTESIAN_POINT('Ctrl Pts',(-17.317963950821,-16.8176412746798,
-1.24121459095794));
#114144=CARTESIAN_POINT('Ctrl Pts',(-17.2495794043259,-16.866311745457,
-1.24538960549146));
#114145=CARTESIAN_POINT('Ctrl Pts',(-17.2241952839492,-16.8843780652956,
-1.24693935725447));
#114146=CARTESIAN_POINT('Ctrl Pts',(-17.1991511792523,-16.902900638027,
-1.24848910901749));
#114147=CARTESIAN_POINT('Ctrl Pts',(-17.1744641548914,-16.9218650419685,
-1.2500388607805));
#114148=CARTESIAN_POINT('Ctrl Pts',(-17.1769962711794,-16.9251779373085,
-0.450077505597091));
#114149=CARTESIAN_POINT('Ctrl Pts',(-16.8637710635621,-17.1646622668181,
-0.469619412639974));
#114150=CARTESIAN_POINT('Ctrl Pts',(-16.0386998885363,-18.1402336475912,
-0.531553255243333));
#114151=CARTESIAN_POINT('Ctrl Pts',(-16.1425599588014,-20.5170161467511,
-0.63587903340717));
#114152=CARTESIAN_POINT('Ctrl Pts',(-18.6471935254001,-21.9777207549249,
-0.763054840088606));
#114153=CARTESIAN_POINT('Ctrl Pts',(-20.8878308446456,-20.8376582577765,
-0.873331792362382));
#114154=CARTESIAN_POINT('Ctrl Pts',(-21.2880301148004,-19.4648724899129,
-0.941216809075682));
#114155=CARTESIAN_POINT('Ctrl Pts',(-21.2904838985449,-18.9506606701336,
-0.966709890228504));
#114156=CARTESIAN_POINT('Origin',(18.734,-18.952,1.76670989022851));
#114157=CARTESIAN_POINT('',(16.1715629797346,-18.9538544393498,-1.0332901097715));
#114158=CARTESIAN_POINT('Ctrl Pts',(20.2957383198016,-16.919032322281,-0.51674866945634));
#114159=CARTESIAN_POINT('Ctrl Pts',(20.9160602511037,-17.401473545096,-0.555987272143906));
#114160=CARTESIAN_POINT('Ctrl Pts',(21.7259565235638,-19.0426368089358,
-0.637617810391948));
#114161=CARTESIAN_POINT('Ctrl Pts',(20.3489602682313,-21.5123500369818,
-0.761640284200471));
#114162=CARTESIAN_POINT('Ctrl Pts',(17.4553335005934,-21.6957541409811,
-0.888816090881904));
#114163=CARTESIAN_POINT('Ctrl Pts',(16.230303771566,-20.0341121451265,-0.979366032738913));
#114164=CARTESIAN_POINT('Ctrl Pts',(16.1706211813573,-19.0694704699527,
-1.02752403903544));
#114165=CARTESIAN_POINT('Ctrl Pts',(16.1715629797346,-18.9538544393498,
-1.0332901097715));
#114166=CARTESIAN_POINT('Ctrl Pts',(16.1715629797346,-18.9538544393498,
-1.0332901097715));
#114167=CARTESIAN_POINT('Ctrl Pts',(16.1775452476667,-18.2194657538418,
-1.06991597459592));
#114168=CARTESIAN_POINT('Ctrl Pts',(16.8944631229174,-16.6248681563667,
-1.14893377498083));
#114169=CARTESIAN_POINT('Ctrl Pts',(19.0022218964003,-16.1791426646111,
-1.24342933787015));
#114170=CARTESIAN_POINT('Ctrl Pts',(20.0455373273649,-16.7324609199408,
-1.30129903593505));
#114171=CARTESIAN_POINT('Ctrl Pts',(20.2916962531305,-16.9242237737287,
-1.31677679843947));
#114172=CARTESIAN_POINT('',(16.174105230784,-18.9506583124956,-0.966709917954191));
#114173=CARTESIAN_POINT('Ctrl Pts',(16.1740003516248,-18.9506582403292,
-0.96670991880675));
#114174=CARTESIAN_POINT('Ctrl Pts',(16.1740492156647,-18.8574284856305,
-0.971325636022637));
#114175=CARTESIAN_POINT('Ctrl Pts',(16.1791950640212,-18.7643768125493,
-0.975941353238524));
#114176=CARTESIAN_POINT('Ctrl Pts',(16.1893550102722,-18.6720323657042,
-0.980557070454411));
#114177=CARTESIAN_POINT('Ctrl Pts',(16.1995507619901,-18.57936248052,-0.985189054282917));
#114178=CARTESIAN_POINT('Ctrl Pts',(16.2147958864483,-18.487405080462,-0.989821038111424));
#114179=CARTESIAN_POINT('Ctrl Pts',(16.234956622384,-18.3966782943254,-0.994453021939931));
#114180=CARTESIAN_POINT('Ctrl Pts',(16.25521618901,-18.3055067530499,-0.999107712387932));
#114181=CARTESIAN_POINT('Ctrl Pts',(16.2804395488529,-18.2155781794355,
-1.00376240283593));
#114182=CARTESIAN_POINT('Ctrl Pts',(16.3104425025438,-18.1273976373283,
-1.00841709328394));
#114183=CARTESIAN_POINT('Ctrl Pts',(16.3297568808632,-18.0706314812951,
-1.01141354667312));
#114184=CARTESIAN_POINT('Ctrl Pts',(16.3510510092264,-18.0145893008769,
-1.0144100000623));
#114185=CARTESIAN_POINT('Ctrl Pts',(16.3742656062904,-17.9594005887852,
-1.01740645345148));
#114186=CARTESIAN_POINT('Ctrl Pts',(16.4066870283893,-17.8823242335553,
-1.02159128939168));
#114187=CARTESIAN_POINT('Ctrl Pts',(16.442949046845,-17.806694695872,-1.02577612533188));
#114188=CARTESIAN_POINT('Ctrl Pts',(16.4829010339938,-17.7329210668517,
-1.02996096127207));
#114189=CARTESIAN_POINT('Ctrl Pts',(16.5227961707087,-17.6592524154088,
-1.03413984232102));
#114190=CARTESIAN_POINT('Ctrl Pts',(16.5663706293486,-17.5874348279767,
-1.03831872336996));
#114191=CARTESIAN_POINT('Ctrl Pts',(16.6134257549123,-17.517857443951,-1.0424976044189));
#114192=CARTESIAN_POINT('Ctrl Pts',(16.6613214140263,-17.4470372170912,
-1.04675113174031));
#114193=CARTESIAN_POINT('Ctrl Pts',(16.7128231258243,-17.378538458199,-1.05100465906173));
#114194=CARTESIAN_POINT('Ctrl Pts',(16.767672421654,-17.312745335637,-1.05525818638315));
#114195=CARTESIAN_POINT('Ctrl Pts',(16.8214616389431,-17.2482238041918,
-1.05942950530122));
#114196=CARTESIAN_POINT('Ctrl Pts',(16.8784698848833,-17.1863046245575,
-1.06360082421929));
#114197=CARTESIAN_POINT('Ctrl Pts',(16.9384107688485,-17.1273193942576,
-1.06777214313735));
#114198=CARTESIAN_POINT('Ctrl Pts',(16.9983315441488,-17.0683539520246,
-1.07194206268243));
#114199=CARTESIAN_POINT('Ctrl Pts',(17.0611826759855,-17.0123208267143,
-1.07611198222751));
#114200=CARTESIAN_POINT('Ctrl Pts',(17.1266402234641,-16.9595154834292,
-1.08028190177259));
#114201=CARTESIAN_POINT('Ctrl Pts',(17.192095441962,-16.9067120189591,-1.08445167295186));
#114202=CARTESIAN_POINT('Ctrl Pts',(17.2601565331721,-16.8571363963205,
-1.08862144413112));
#114203=CARTESIAN_POINT('Ctrl Pts',(17.3304667893585,-16.8110435486385,
-1.09279121531039));
#114204=CARTESIAN_POINT('Ctrl Pts',(17.4032413988251,-16.7633351605427,
-1.09710713571227));
#114205=CARTESIAN_POINT('Ctrl Pts',(17.4784253279814,-16.7193585145734,
-1.10142305611414));
#114206=CARTESIAN_POINT('Ctrl Pts',(17.5555924665286,-16.6793461141085,
-1.10573897651602));
#114207=CARTESIAN_POINT('Ctrl Pts',(17.6302537175965,-16.6406330565404,
-1.10991474385404));
#114208=CARTESIAN_POINT('Ctrl Pts',(17.7067708977367,-16.6056308716597,
-1.11409051119206));
#114209=CARTESIAN_POINT('Ctrl Pts',(17.7847367550311,-16.5745014633546,
-1.11826627853008));
#114210=CARTESIAN_POINT('Ctrl Pts',(17.8666278144111,-16.5418048405963,
-1.12265227546388));
#114211=CARTESIAN_POINT('Ctrl Pts',(17.950116694982,-16.5133813683478,-1.12703827239769));
#114212=CARTESIAN_POINT('Ctrl Pts',(18.0347145687176,-16.4893591643124,
-1.13142426933149));
#114213=CARTESIAN_POINT('Ctrl Pts',(18.1193124424532,-16.465336960277,-1.1358102662653));
#114214=CARTESIAN_POINT('Ctrl Pts',(18.2050187273114,-16.445716079792,-1.1401962631991));
#114215=CARTESIAN_POINT('Ctrl Pts',(18.2913357970735,-16.4305622348653,
-1.14458226013291));
#114216=CARTESIAN_POINT('Ctrl Pts',(18.3778108630074,-16.4153806520938,
-1.14897628526701));
#114217=CARTESIAN_POINT('Ctrl Pts',(18.4652367601027,-16.4046231872553,
-1.15337031040112));
#114218=CARTESIAN_POINT('Ctrl Pts',(18.5531205108655,-16.398398110431,-1.15776433553522));
#114219=CARTESIAN_POINT('Ctrl Pts',(18.6366787085168,-16.39247942586,-1.16194209100712));
#114220=CARTESIAN_POINT('Ctrl Pts',(18.7206502243009,-16.3906576252416,
-1.16611984647902));
#114221=CARTESIAN_POINT('Ctrl Pts',(18.8046002870634,-16.3929737009037,
-1.17029760195092));
#114222=CARTESIAN_POINT('Ctrl Pts',(18.8884688502721,-16.3952875280966,
-1.17447130161636));
#114223=CARTESIAN_POINT('Ctrl Pts',(18.9723155446172,-16.4017312428622,
-1.1786450012818));
#114224=CARTESIAN_POINT('Ctrl Pts',(19.0557029730719,-16.4122938758359,
-1.18281870094723));
#114225=CARTESIAN_POINT('Ctrl Pts',(19.1390344624023,-16.422849423036,-1.18698960075292));
#114226=CARTESIAN_POINT('Ctrl Pts',(19.2219068427816,-16.4375183423304,
-1.19116050055861));
#114227=CARTESIAN_POINT('Ctrl Pts',(19.3038865859859,-16.4562377358584,
-1.1953314003643));
#114228=CARTESIAN_POINT('Ctrl Pts',(19.3858359242349,-16.4749501866673,
-1.19950075325099));
#114229=CARTESIAN_POINT('Ctrl Pts',(19.4668928355199,-16.4977100230749,
-1.20367010613769));
#114230=CARTESIAN_POINT('Ctrl Pts',(19.5466340988466,-16.5244032827935,
-1.20783945902438));
#114231=CARTESIAN_POINT('Ctrl Pts',(19.6263975218472,-16.5511039604273,
-1.21200997055212));
#114232=CARTESIAN_POINT('Ctrl Pts',(19.7048441281799,-16.5817401045136,
-1.21618048207985));
#114233=CARTESIAN_POINT('Ctrl Pts',(19.7815668566494,-16.61614818945,-1.22035099360759));
#114234=CARTESIAN_POINT('Ctrl Pts',(19.8583020478613,-16.650561863592,-1.22452218258792));
#114235=CARTESIAN_POINT('Ctrl Pts',(19.9333123891112,-16.6887484987226,
-1.22869337156825));
#114236=CARTESIAN_POINT('Ctrl Pts',(20.0062135173125,-16.7304976330493,
-1.23286456054858));
#114237=CARTESIAN_POINT('Ctrl Pts',(20.0791815041405,-16.7722850560811,
-1.23703957498366));
#114238=CARTESIAN_POINT('Ctrl Pts',(20.1500360249586,-16.8176412586702,
-1.24121458941875));
#114239=CARTESIAN_POINT('Ctrl Pts',(20.2184205708046,-16.8663117277569,
-1.24538960385383));
#114240=CARTESIAN_POINT('Ctrl Pts',(20.2438047145168,-16.8843780637479,
-1.2469393570197));
#114241=CARTESIAN_POINT('Ctrl Pts',(20.2688488419368,-16.902900653468,-1.24848911018556));
#114242=CARTESIAN_POINT('Ctrl Pts',(20.293535888361,-16.9218650751948,-1.25003886335143));
#114243=CARTESIAN_POINT('Ctrl Pts',(20.2910039261765,-16.9251777670034,
-0.450077510764929));
#114244=CARTESIAN_POINT('Ctrl Pts',(20.6042291142437,-17.1646622078131,
-0.469619416085199));
#114245=CARTESIAN_POINT('Ctrl Pts',(21.4293002690834,-18.1402340273379,
-0.531553256965945));
#114246=CARTESIAN_POINT('Ctrl Pts',(21.3254401485204,-20.5170159135665,
-0.635879033407171));
#114247=CARTESIAN_POINT('Ctrl Pts',(18.8208065113563,-21.977721108989,-0.763054840088605));
#114248=CARTESIAN_POINT('Ctrl Pts',(16.5801690201362,-20.8376582933814,
-0.873331792362383));
#114249=CARTESIAN_POINT('Ctrl Pts',(16.1799697387475,-19.4648724906692,
-0.941216809075683));
#114250=CARTESIAN_POINT('Ctrl Pts',(16.1775159588735,-18.9506606593868,
-0.966709890228505));
#114251=CARTESIAN_POINT('Origin',(18.734,19.211,1.76670989022852));
#114252=CARTESIAN_POINT('',(16.1715629762874,19.209145560805,-1.0332901097715));
#114253=CARTESIAN_POINT('Ctrl Pts',(20.2957383200499,21.2439676837843,-0.516748669299169));
#114254=CARTESIAN_POINT('Ctrl Pts',(20.9160602538759,20.7615264607868,-0.555987272039123));
#114255=CARTESIAN_POINT('Ctrl Pts',(21.725956527216,19.1203631895649,-0.637617810339557));
#114256=CARTESIAN_POINT('Ctrl Pts',(20.3489602709871,16.6506499609975,-0.76164028420047));
#114257=CARTESIAN_POINT('Ctrl Pts',(17.4553334985585,16.4672458544258,-0.888816090881905));
#114258=CARTESIAN_POINT('Ctrl Pts',(16.2303037681755,18.1288878534983,-0.979366032738912));
#114259=CARTESIAN_POINT('Ctrl Pts',(16.1706211779077,19.0935295300429,-1.02752403903544));
#114260=CARTESIAN_POINT('Ctrl Pts',(16.1715629762874,19.209145560805,-1.0332901097715));
#114261=CARTESIAN_POINT('Ctrl Pts',(16.1715629762874,19.209145560805,-1.0332901097715));
#114262=CARTESIAN_POINT('Ctrl Pts',(16.1775452442342,19.9435342473242,-1.06991597459592));
#114263=CARTESIAN_POINT('Ctrl Pts',(16.8944631203331,21.5381318465523,-1.14893377498083));
#114264=CARTESIAN_POINT('Ctrl Pts',(19.0022218955,21.9838573389643,-1.24342933781265));
#114265=CARTESIAN_POINT('Ctrl Pts',(20.0455373270949,21.4305390842377,-1.30129903582005));
#114266=CARTESIAN_POINT('Ctrl Pts',(20.2916962525238,21.2387762312158,-1.31677679826698));
#114267=CARTESIAN_POINT('',(16.1741052276289,19.2123416889722,-0.966709917954053));
#114268=CARTESIAN_POINT('Ctrl Pts',(16.1740003516256,19.2123417611365,-0.966709918806587));
#114269=CARTESIAN_POINT('Ctrl Pts',(16.174049215721,19.3055715198376,-0.971325636241826));
#114270=CARTESIAN_POINT('Ctrl Pts',(16.17919506457,19.3986231969093,-0.975941353677064));
#114271=CARTESIAN_POINT('Ctrl Pts',(16.1893550117453,19.490967647685,-0.980557071112303));
#114272=CARTESIAN_POINT('Ctrl Pts',(16.1995507644016,19.5836375369126,-0.985189055165875));
#114273=CARTESIAN_POINT('Ctrl Pts',(16.2147958902436,19.6755949409525,-0.989821039219448));
#114274=CARTESIAN_POINT('Ctrl Pts',(16.2349566280026,19.7663217309596,-0.99445302327302));
#114275=CARTESIAN_POINT('Ctrl Pts',(16.2552161964654,19.8574932761445,-0.99910771394821));
#114276=CARTESIAN_POINT('Ctrl Pts',(16.2804395585911,19.9474218535553,-1.0037624046234));
#114277=CARTESIAN_POINT('Ctrl Pts',(16.3104425150043,20.0356023992939,-1.00841709529859));
#114278=CARTESIAN_POINT('Ctrl Pts',(16.3297568898048,20.0923685421719,-1.01141354801622));
#114279=CARTESIAN_POINT('Ctrl Pts',(16.3510510137503,20.1484107097619,-1.01441000073385));
#114280=CARTESIAN_POINT('Ctrl Pts',(16.3742656055452,20.2035994094432,-1.01740645345148));
#114281=CARTESIAN_POINT('Ctrl Pts',(16.4066870270799,20.2806757634937,-1.0215912893308));
#114282=CARTESIAN_POINT('Ctrl Pts',(16.4429490448682,20.3563053000825,-1.02577612521011));
#114283=CARTESIAN_POINT('Ctrl Pts',(16.4829010312601,20.4300789281004,-1.02996096108943));
#114284=CARTESIAN_POINT('Ctrl Pts',(16.5227961672129,20.5037475785304,-1.03413984207691));
#114285=CARTESIAN_POINT('Ctrl Pts',(16.5663706250003,20.575565165042,-1.03831872306438));
#114286=CARTESIAN_POINT('Ctrl Pts',(16.6134257496346,20.6451425482453,-1.04249760405186));
#114287=CARTESIAN_POINT('Ctrl Pts',(16.6613214086794,20.7159627755642,-1.04675113138857));
#114288=CARTESIAN_POINT('Ctrl Pts',(16.7128231204605,20.7844615349321,-1.05100465872528));
#114289=CARTESIAN_POINT('Ctrl Pts',(16.7676724163246,20.8502546579702,-1.05525818606199));
#114290=CARTESIAN_POINT('Ctrl Pts',(16.8214616326485,20.9147761886841,-1.05942950491759));
#114291=CARTESIAN_POINT('Ctrl Pts',(16.878469877553,20.9766953676843,-1.06360082377319));
#114292=CARTESIAN_POINT('Ctrl Pts',(16.9384107604234,21.0356805974517,-1.06777214262878));
#114293=CARTESIAN_POINT('Ctrl Pts',(16.9983315346257,21.0946460391488,-1.07194206211116));
#114294=CARTESIAN_POINT('Ctrl Pts',(17.0611826653049,21.150679164025,-1.07611198159354));
#114295=CARTESIAN_POINT('Ctrl Pts',(17.1266402115777,21.2034845069819,-1.08028190107591));
#114296=CARTESIAN_POINT('Ctrl Pts',(17.1920954288672,21.2562879711218,-1.08445167219232));
#114297=CARTESIAN_POINT('Ctrl Pts',(17.2601565188203,21.3058635935363,-1.08862144330872));
#114298=CARTESIAN_POINT('Ctrl Pts',(17.3304667737115,21.3519564411039,-1.09279121442513));
#114299=CARTESIAN_POINT('Ctrl Pts',(17.4032413841786,21.399664830616,-1.09710713490077));
#114300=CARTESIAN_POINT('Ctrl Pts',(17.4784253144497,21.4436414778789,-1.10142305537642));
#114301=CARTESIAN_POINT('Ctrl Pts',(17.5555924541958,21.4836538794968,-1.10573897585207));
#114302=CARTESIAN_POINT('Ctrl Pts',(17.6302537040283,21.5223669369384,-1.10991474312749));
#114303=CARTESIAN_POINT('Ctrl Pts',(17.7067708828925,21.5573691217994,-1.11409051040291));
#114304=CARTESIAN_POINT('Ctrl Pts',(17.7847367388801,21.5884985301968,-1.11826627767833));
#114305=CARTESIAN_POINT('Ctrl Pts',(17.8666278007655,21.6211951546004,-1.12265227475409));
#114306=CARTESIAN_POINT('Ctrl Pts',(17.9501166839591,21.6496186282125,-1.12703827182985));
#114307=CARTESIAN_POINT('Ctrl Pts',(18.0347145603764,21.6736408333191,-1.13142426890562));
#114308=CARTESIAN_POINT('Ctrl Pts',(18.1193124367938,21.6976630384256,-1.13581026598138));
#114309=CARTESIAN_POINT('Ctrl Pts',(18.2050187243926,21.7172839196893,-1.14019626305714));
#114310=CARTESIAN_POINT('Ctrl Pts',(18.2913357968955,21.7324377651034,-1.1445822601329));
#114311=CARTESIAN_POINT('Ctrl Pts',(18.3778108626164,21.7476193478439,-1.14897628525888));
#114312=CARTESIAN_POINT('Ctrl Pts',(18.4652367595084,21.7583768126755,-1.15337031038486));
#114313=CARTESIAN_POINT('Ctrl Pts',(18.55312051008,21.7646018895134,-1.15776433551083));
#114314=CARTESIAN_POINT('Ctrl Pts',(18.6366787074649,21.7705205740913,-1.16194209097077));
#114315=CARTESIAN_POINT('Ctrl Pts',(18.7206502229926,21.7723423747436,-1.16611984643071));
#114316=CARTESIAN_POINT('Ctrl Pts',(18.8046002855114,21.7700262991391,-1.17029760189066));
#114317=CARTESIAN_POINT('Ctrl Pts',(18.8884688484699,21.7677124720041,-1.17447130154382));
#114318=CARTESIAN_POINT('Ctrl Pts',(18.9723155425776,21.7612687573207,-1.17864500119699));
#114319=CARTESIAN_POINT('Ctrl Pts',(19.0557029708096,21.7507061244507,-1.18281870085015));
#114320=CARTESIAN_POINT('Ctrl Pts',(19.1390344599114,21.7401505773549,-1.18698960064328));
#114321=CARTESIAN_POINT('Ctrl Pts',(19.2219068400769,21.7254816581869,-1.1911605004364));
#114322=CARTESIAN_POINT('Ctrl Pts',(19.3038865830838,21.7067622648043,-1.19533140022953));
#114323=CARTESIAN_POINT('Ctrl Pts',(19.3858359211298,21.688049814142,-1.19950075310337));
#114324=CARTESIAN_POINT('Ctrl Pts',(19.4668928322285,21.6652899779005,-1.20367010597722));
#114325=CARTESIAN_POINT('Ctrl Pts',(19.5466340953869,21.6385967183646,-1.20783945885106));
#114326=CARTESIAN_POINT('Ctrl Pts',(19.6263975182123,21.6118960409159,-1.21200997036559));
#114327=CARTESIAN_POINT('Ctrl Pts',(19.704844124388,21.581259897032,-1.21618048188011));
#114328=CARTESIAN_POINT('Ctrl Pts',(19.7815668527197,21.5468518123123,-1.22035099339464));
#114329=CARTESIAN_POINT('Ctrl Pts',(19.8583020437901,21.5124381383889,-1.22452218236154));
#114330=CARTESIAN_POINT('Ctrl Pts',(19.9333123849178,21.4742515034917,-1.22869337132845));
#114331=CARTESIAN_POINT('Ctrl Pts',(20.0062135130172,21.4325023694105,-1.23286456029535));
#114332=CARTESIAN_POINT('Ctrl Pts',(20.0791814997391,21.3907149466269,-1.23703957471676));
#114333=CARTESIAN_POINT('Ctrl Pts',(20.1500360204715,21.3453587442986,-1.24121458913816));
#114334=CARTESIAN_POINT('Ctrl Pts',(20.218420566253,21.2966882754825,-1.24538960355956));
#114335=CARTESIAN_POINT('Ctrl Pts',(20.2438047105659,21.2786219391475,-1.24693935675848));
#114336=CARTESIAN_POINT('Ctrl Pts',(20.2688488385727,21.2600993490623,-1.2484891099574));
#114337=CARTESIAN_POINT('Ctrl Pts',(20.2935358855687,21.2411349269503,-1.25003886315632));
#114338=CARTESIAN_POINT('Ctrl Pts',(20.2910039445873,21.2378222631174,-0.450077510930245));
#114339=CARTESIAN_POINT('Ctrl Pts',(20.6042291338676,20.9983378060478,-0.46961941619541));
#114340=CARTESIAN_POINT('Ctrl Pts',(21.4293002909665,20.0227659246052,-0.53155325702105));
#114341=CARTESIAN_POINT('Ctrl Pts',(21.3254401632976,17.6459841184673,-0.635879033407171));
#114342=CARTESIAN_POINT('Ctrl Pts',(18.8208065164127,16.1852788423107,-0.763054840088604));
#114343=CARTESIAN_POINT('Ctrl Pts',(16.5801690015235,17.3253417016998,-0.873331792362383));
#114344=CARTESIAN_POINT('Ctrl Pts',(16.1799697185864,18.6981275092202,-0.941216809075682));
#114345=CARTESIAN_POINT('Ctrl Pts',(16.1775159392447,19.2123393420905,-0.966709890228504));
#114346=CARTESIAN_POINT('Origin',(-18.734,19.211,1.76670989022852));
#114347=CARTESIAN_POINT('',(-21.2964371839251,19.2091455679848,-1.0332901097715));
#114348=CARTESIAN_POINT('Ctrl Pts',(-17.1722616682727,21.2439679654049,
-0.516748662007315));
#114349=CARTESIAN_POINT('Ctrl Pts',(-16.5519396172804,20.761526733893,-0.555987267177887));
#114350=CARTESIAN_POINT('Ctrl Pts',(-15.7420433029967,19.120363119997,-0.637617807908939));
#114351=CARTESIAN_POINT('Ctrl Pts',(-17.1190396009992,16.6506498669621,
-0.761640284200469));
#114352=CARTESIAN_POINT('Ctrl Pts',(-20.0126665959802,16.4672456410459,
-0.888816090881905));
#114353=CARTESIAN_POINT('Ctrl Pts',(-21.2376963893991,18.1288877895766,
-0.979366032738913));
#114354=CARTESIAN_POINT('Ctrl Pts',(-21.2973789824122,19.0935295298239,
-1.02752403903544));
#114355=CARTESIAN_POINT('Ctrl Pts',(-21.2964371839251,19.2091455679848,
-1.0332901097715));
#114356=CARTESIAN_POINT('Ctrl Pts',(-21.2964371839251,19.2091455679848,
-1.0332901097715));
#114357=CARTESIAN_POINT('Ctrl Pts',(-21.2904549152958,19.943534301501,-1.06991597459592));
#114358=CARTESIAN_POINT('Ctrl Pts',(-20.5735369997583,21.5381319822354,
-1.14893377498083));
#114359=CARTESIAN_POINT('Ctrl Pts',(-18.4657781462453,21.983857505142,-1.24342933514492));
#114360=CARTESIAN_POINT('Ctrl Pts',(-17.4224626852965,21.4305392783363,
-1.30129903048459));
#114361=CARTESIAN_POINT('Ctrl Pts',(-17.1763037754663,21.2387764608407,
-1.31677679026378));
#114362=CARTESIAN_POINT('',(-21.2938947647296,19.2123416854176,-0.966709917954385));
#114363=CARTESIAN_POINT('Ctrl Pts',(-21.2939996483763,19.212341757587,-0.96670991880698));
#114364=CARTESIAN_POINT('Ctrl Pts',(-21.2939507844152,19.3055715065957,
-0.971325635711016));
#114365=CARTESIAN_POINT('Ctrl Pts',(-21.2888049367591,19.3986231740038,
-0.975941352615052));
#114366=CARTESIAN_POINT('Ctrl Pts',(-21.2786449918221,19.4909676152607,
-0.980557069519088));
#114367=CARTESIAN_POINT('Ctrl Pts',(-21.2684492414382,19.5836374946964,
-0.985189053027621));
#114368=CARTESIAN_POINT('Ctrl Pts',(-21.2532041189474,19.6755948890935,
-0.989821036536154));
#114369=CARTESIAN_POINT('Ctrl Pts',(-21.233043385604,19.7663216697276,-0.994453020044687));
#114370=CARTESIAN_POINT('Ctrl Pts',(-21.2127838215892,19.8574932054453,
-0.999107710169702));
#114371=CARTESIAN_POINT('Ctrl Pts',(-21.1875604649916,19.9474217736623,
-1.00376240029472));
#114372=CARTESIAN_POINT('Ctrl Pts',(-21.1575575151709,20.035602310607,-1.00841709041973));
#114373=CARTESIAN_POINT('Ctrl Pts',(-21.1382431318488,20.0923684853426,
-1.01141354476365));
#114374=CARTESIAN_POINT('Ctrl Pts',(-21.1169489972049,20.1484106839985,
-1.01440999910756));
#114375=CARTESIAN_POINT('Ctrl Pts',(-21.09373439265,20.2035994137337,-1.01740645345148));
#114376=CARTESIAN_POINT('Ctrl Pts',(-21.0613129697488,20.2806757706407,
-1.02159128947824));
#114377=CARTESIAN_POINT('Ctrl Pts',(-21.0250509503441,20.3563053098801,
-1.02577612550499));
#114378=CARTESIAN_POINT('Ctrl Pts',(-20.9850989621192,20.4300789403257,
-1.02996096153175));
#114379=CARTESIAN_POINT('Ctrl Pts',(-20.9452038243207,20.5037475932088,
-1.03413984266809));
#114380=CARTESIAN_POINT('Ctrl Pts',(-20.9016293644687,20.5755651819498,
-1.03831872380443));
#114381=CARTESIAN_POINT('Ctrl Pts',(-20.8545742375835,20.6451425671449,
-1.04249760494077));
#114382=CARTESIAN_POINT('Ctrl Pts',(-20.806678578371,20.7159627933518,-1.04675113224044));
#114383=CARTESIAN_POINT('Ctrl Pts',(-20.7551768665491,20.7844615515677,
-1.05100465954011));
#114384=CARTESIAN_POINT('Ctrl Pts',(-20.7003275707683,20.8502546734527,
-1.05525818683978));
#114385=CARTESIAN_POINT('Ctrl Pts',(-20.6465383521068,20.9147762059375,
-1.05942950584667));
#114386=CARTESIAN_POINT('Ctrl Pts',(-20.5895301046941,20.9766953864735,
-1.06360082485355));
#114387=CARTESIAN_POINT('Ctrl Pts',(-20.5295892191724,21.0356806175306,
-1.06777214386044));
#114388=CARTESIAN_POINT('Ctrl Pts',(-20.4696684423108,21.0946460605256,
-1.07194206349468));
#114389=CARTESIAN_POINT('Ctrl Pts',(-20.4068173088285,21.150679186453,-1.07611198312891));
#114390=CARTESIAN_POINT('Ctrl Pts',(-20.3413597596352,21.2034845302048,
-1.08028190276314));
#114391=CARTESIAN_POINT('Ctrl Pts',(-20.2759045394194,21.2562879951442,
-1.08445167403178));
#114392=CARTESIAN_POINT('Ctrl Pts',(-20.2078434464222,21.3058636181013,
-1.08862144530041));
#114393=CARTESIAN_POINT('Ctrl Pts',(-20.1375331883945,21.3519564659458,
-1.09279121656905));
#114394=CARTESIAN_POINT('Ctrl Pts',(-20.0647585803504,21.3996648520279,
-1.09710713686604));
#114395=CARTESIAN_POINT('Ctrl Pts',(-19.9895746527792,21.443641496158,-1.10142305716302));
#114396=CARTESIAN_POINT('Ctrl Pts',(-19.9124075159367,21.4836538949836,
-1.10573897746001));
#114397=CARTESIAN_POINT('Ctrl Pts',(-19.8377462631121,21.5223669527316,
-1.10991474488704));
#114398=CARTESIAN_POINT('Ctrl Pts',(-19.7612290811577,21.5573691376402,
-1.11409051231407));
#114399=CARTESIAN_POINT('Ctrl Pts',(-19.6832632220051,21.5884985458142,
-1.1182662797411));
#114400=CARTESIAN_POINT('Ctrl Pts',(-19.6013721661874,21.621195166233,-1.12265227647306));
#114401=CARTESIAN_POINT('Ctrl Pts',(-19.5178832893455,21.6496186365428,
-1.12703827320503));
#114402=CARTESIAN_POINT('Ctrl Pts',(-19.4332854194228,21.6736408390552,
-1.131424269937));
#114403=CARTESIAN_POINT('Ctrl Pts',(-19.3486875495001,21.6976630415676,
-1.13581026666897));
#114404=CARTESIAN_POINT('Ctrl Pts',(-19.2629812685386,21.7172839209455,
-1.14019626340094));
#114405=CARTESIAN_POINT('Ctrl Pts',(-19.1766642026735,21.7324377651791,
-1.1445822601329));
#114406=CARTESIAN_POINT('Ctrl Pts',(-19.0901891434539,21.7476193467629,
-1.148976284922));
#114407=CARTESIAN_POINT('Ctrl Pts',(-19.0027632532416,21.7583768110981,
-1.15337030971109));
#114408=CARTESIAN_POINT('Ctrl Pts',(-18.9148795094127,21.7646018881326,
-1.15776433450019));
#114409=CARTESIAN_POINT('Ctrl Pts',(-18.831321311443,21.770520573393,-1.16194208998959));
#114410=CARTESIAN_POINT('Ctrl Pts',(-18.7473497953179,21.7723423746674,
-1.16611984547899));
#114411=CARTESIAN_POINT('Ctrl Pts',(-18.663399732195,21.7700262996276,-1.1702976009684));
#114412=CARTESIAN_POINT('Ctrl Pts',(-18.5795311686207,21.7677124730563,
-1.1744713006516));
#114413=CARTESIAN_POINT('Ctrl Pts',(-18.4956844738905,21.7612687588782,
-1.1786450003348));
#114414=CARTESIAN_POINT('Ctrl Pts',(-18.4122970450345,21.7507061264576,
-1.182818700018));
#114415=CARTESIAN_POINT('Ctrl Pts',(-18.328965555298,21.7401505798097,-1.1869895998417));
#114416=CARTESIAN_POINT('Ctrl Pts',(-18.2460931744964,21.7254816610328,
-1.19116049966539));
#114417=CARTESIAN_POINT('Ctrl Pts',(-18.1641134308566,21.7067622679875,
-1.19533139948908));
#114418=CARTESIAN_POINT('Ctrl Pts',(-18.082164092168,21.68804981766,-1.199500752394));
#114419=CARTESIAN_POINT('Ctrl Pts',(-18.0011071804304,21.6652899816987,
-1.20367010529891));
#114420=CARTESIAN_POINT('Ctrl Pts',(-17.921365916641,21.6385967223909,-1.20783945820382));
#114421=CARTESIAN_POINT('Ctrl Pts',(-17.8416024931822,21.6118960451696,
-1.21200996974954));
#114422=CARTESIAN_POINT('Ctrl Pts',(-17.7631558863812,21.581259901461,-1.21618048129526));
#114423=CARTESIAN_POINT('Ctrl Pts',(-17.6864331574362,21.546851816867,-1.22035099284098));
#114424=CARTESIAN_POINT('Ctrl Pts',(-17.6096979657455,21.5124381430661,
-1.22452218183947));
#114425=CARTESIAN_POINT('Ctrl Pts',(-17.5346876240098,21.4742515082411,
-1.22869337083796));
#114426=CARTESIAN_POINT('Ctrl Pts',(-17.4617864953189,21.4325023741844,
-1.23286455983645));
#114427=CARTESIAN_POINT('Ctrl Pts',(-17.3888185080204,21.3907149514342,
-1.23703957428859));
#114428=CARTESIAN_POINT('Ctrl Pts',(-17.3179639867267,21.3453587490929,
-1.24121458874073));
#114429=CARTESIAN_POINT('Ctrl Pts',(-17.2495794404032,21.2966882802198,
-1.24538960319287));
#114430=CARTESIAN_POINT('Ctrl Pts',(-17.2241953382174,21.2786219739895,
-1.24693935381897));
#114431=CARTESIAN_POINT('Ctrl Pts',(-17.1991512512063,21.2600994155247,
-1.24848910444507));
#114432=CARTESIAN_POINT('Ctrl Pts',(-17.1744642439897,21.2411350264762,
-1.25003885507116));
#114433=CARTESIAN_POINT('Ctrl Pts',(-17.1769962363369,21.2378222944355,
-0.450077502023298));
#114434=CARTESIAN_POINT('Ctrl Pts',(-16.8637709891942,20.998337861822,-0.469619410257445));
#114435=CARTESIAN_POINT('Ctrl Pts',(-16.0386997591895,20.0227661055849,
-0.531553254052069));
#114436=CARTESIAN_POINT('Ctrl Pts',(-16.1425598724776,17.6459840408836,
-0.635879033407169));
#114437=CARTESIAN_POINT('Ctrl Pts',(-18.6471934958306,16.1852789602342,
-0.763054840088606));
#114438=CARTESIAN_POINT('Ctrl Pts',(-20.8878309534133,17.3253417136014,
-0.873331792362382));
#114439=CARTESIAN_POINT('Ctrl Pts',(-21.2880302326024,18.6981275094852,
-0.941216809075682));
#114440=CARTESIAN_POINT('Ctrl Pts',(-21.2904840132329,19.212339338513,-0.966709890228504));
#114441=CARTESIAN_POINT('Origin',(26.8463464956315,10.1295,-7.));
#114442=CARTESIAN_POINT('',(21.5963464956316,10.1298829051514,-12.098999985623));
#114443=CARTESIAN_POINT('Ctrl Pts',(22.5651720735026,6.08350804222181,-3.89745662547247));
#114444=CARTESIAN_POINT('Ctrl Pts',(22.5448385294137,6.3478784765494,-3.55278409554048));
#114445=CARTESIAN_POINT('Ctrl Pts',(22.4857231036888,7.24322563422365,-2.64786715344243));
#114446=CARTESIAN_POINT('Ctrl Pts',(22.3878257963277,9.21233876997001,-1.77459149097018));
#114447=CARTESIAN_POINT('Ctrl Pts',(22.2714801514196,11.7661169025298,-1.95345839105347));
#114448=CARTESIAN_POINT('Ctrl Pts',(22.1551345065114,13.9387381504676,-3.30737374765752));
#114449=CARTESIAN_POINT('Ctrl Pts',(22.0387888616032,15.2245708351663,-5.52111016209781));
#114450=CARTESIAN_POINT('Ctrl Pts',(21.922443216695,15.3236941270903,-8.07916377113051));
#114451=CARTESIAN_POINT('Ctrl Pts',(21.8060975717868,14.2141213326594,-10.3860101586105));
#114452=CARTESIAN_POINT('Ctrl Pts',(21.6973986661381,12.2874582761103,-11.804511236185));
#114453=CARTESIAN_POINT('Ctrl Pts',(21.6274816421253,10.7948600303933,-12.0984964626806));
#114454=CARTESIAN_POINT('Ctrl Pts',(21.5963464997487,10.1298830029783,-12.0991317633798));
#114455=CARTESIAN_POINT('Ctrl Pts',(21.5963464956316,10.1298829051514,-12.098999985623));
#114456=CARTESIAN_POINT('Ctrl Pts',(21.5886997577445,9.96656989073889,-12.0990122494776));
#114457=CARTESIAN_POINT('Ctrl Pts',(21.5810530198574,9.80325714346398,-12.0911738586918));
#114458=CARTESIAN_POINT('Ctrl Pts',(21.5734062819704,9.64065518488774,-12.0755129540508));
#114459=CARTESIAN_POINT('Ctrl Pts',(21.5666845761133,9.49772331596717,-12.0617465616352));
#114460=CARTESIAN_POINT('Ctrl Pts',(21.5599628702561,9.35531775886811,-12.0419328173513));
#114461=CARTESIAN_POINT('Ctrl Pts',(21.553241164399,9.21397363696974,-12.0161352133487));
#114462=CARTESIAN_POINT('Ctrl Pts',(21.5465211079346,9.07266419852288,-11.9903439396408));
#114463=CARTESIAN_POINT('Ctrl Pts',(21.5398010514701,8.93241603785332,-11.9585717981774));
#114464=CARTESIAN_POINT('Ctrl Pts',(21.5330809950056,8.79375579412643,-11.9209336935662));
#114465=CARTESIAN_POINT('Ctrl Pts',(21.5263596207543,8.65506835945939,-11.8832882082133));
#114466=CARTESIAN_POINT('Ctrl Pts',(21.5196382465029,8.51796982061406,-11.8397745520151));
#114467=CARTESIAN_POINT('Ctrl Pts',(21.5129168722516,8.38297363001403,-11.790558071764));
#114468=CARTESIAN_POINT('Ctrl Pts',(21.5061950124626,8.24796768757988,-11.7413380362204));
#114469=CARTESIAN_POINT('Ctrl Pts',(21.4994731526736,8.11506473991455,-11.6864144868448));
#114470=CARTESIAN_POINT('Ctrl Pts',(21.4927512928847,7.9847596072539,-11.6260014751104));
#114471=CARTESIAN_POINT('Ctrl Pts',(21.4860249738077,7.85436803004691,-11.5655483853277));
#114472=CARTESIAN_POINT('Ctrl Pts',(21.4792986547307,7.72657804372845,-11.4995987153755));
#114473=CARTESIAN_POINT('Ctrl Pts',(21.4725723356537,7.60186164562879,-11.4284134122179));
#114474=CARTESIAN_POINT('Ctrl Pts',(21.4674017694565,7.50599132118198,-11.3736927963763));
#114475=CARTESIAN_POINT('Ctrl Pts',(21.4622312032594,7.41193676657903,-11.3158793604137));
#114476=CARTESIAN_POINT('Ctrl Pts',(21.4570606370622,7.31990104245665,-11.2551092462793));
#114477=CARTESIAN_POINT('Ctrl Pts',(21.4497821926166,7.19034522990356,-11.1695650557955));
#114478=CARTESIAN_POINT('Ctrl Pts',(21.4425037481711,7.06471083663906,-11.0781083746355));
#114479=CARTESIAN_POINT('Ctrl Pts',(21.4352253037255,6.94350501939066,-10.9811100190188));
#114480=CARTESIAN_POINT('Ctrl Pts',(21.4279477400291,6.82231386900175,-10.8841234009679));
#114481=CARTESIAN_POINT('Ctrl Pts',(21.4206701763327,6.70555042157178,-10.7815966068709));
#114482=CARTESIAN_POINT('Ctrl Pts',(21.4133926126363,6.59368928068819,-10.6739411477594));
#114483=CARTESIAN_POINT('Ctrl Pts',(21.4061193938006,6.48189492329082,-10.5663499612524));
#114484=CARTESIAN_POINT('Ctrl Pts',(21.3988461749649,6.374997207616,-10.4536364025609));
#114485=CARTESIAN_POINT('Ctrl Pts',(21.3915729561292,6.27343466828419,-10.3362495646368));
#114486=CARTESIAN_POINT('Ctrl Pts',(21.3843045826288,6.17193978875607,-10.2189409284834));
#114487=CARTESIAN_POINT('Ctrl Pts',(21.3770362091284,6.07577315665127,-10.0969654188858));
#114488=CARTESIAN_POINT('Ctrl Pts',(21.369767835628,5.98533451912964,-9.97080687140086));
#114489=CARTESIAN_POINT('Ctrl Pts',(21.362508451111,5.89500772938303,-9.84480434741678));
#114490=CARTESIAN_POINT('Ctrl Pts',(21.3552490665939,5.81039493847136,-9.71462931976104));
#114491=CARTESIAN_POINT('Ctrl Pts',(21.3479896820768,5.73185403598033,-9.58079657763674));
#114492=CARTESIAN_POINT('Ctrl Pts',(21.3455647854359,5.70561853761555,-9.53609160766829));
#114493=CARTESIAN_POINT('Ctrl Pts',(21.3431398887949,5.68006019676905,-9.49097876732916));
#114494=CARTESIAN_POINT('Ctrl Pts',(21.340714992154,5.65519129922816,-9.44547800035033));
#114495=CARTESIAN_POINT('Ctrl Pts',(21.3339842151457,5.58616278850139,-9.31918168277893));
#114496=CARTESIAN_POINT('Ctrl Pts',(21.3272534381374,5.5224727999895,-9.18993727191009));
#114497=CARTESIAN_POINT('Ctrl Pts',(21.320522661129,5.46436371111823,-9.05822846306196));
#114498=CARTESIAN_POINT('Ctrl Pts',(21.3137921028903,5.40625651095962,-8.92652393512925));
#114499=CARTESIAN_POINT('Ctrl Pts',(21.3070615446517,5.35372999568267,-8.79235550376611));
#114500=CARTESIAN_POINT('Ctrl Pts',(21.300330986413,5.30697886832862,-8.65622792350057));
#114501=CARTESIAN_POINT('Ctrl Pts',(21.2935969859559,5.26020383098296,-8.52003072332451));
#114502=CARTESIAN_POINT('Ctrl Pts',(21.2868629854988,5.21921020433081,-8.38187271779159));
#114503=CARTESIAN_POINT('Ctrl Pts',(21.2801289850417,5.18414331691865,-8.24227544333075));
#114504=CARTESIAN_POINT('Ctrl Pts',(21.2733933187736,5.14906775489954,-8.10264363625022));
#114505=CARTESIAN_POINT('Ctrl Pts',(21.2666576525055,5.11992193614115,-7.96157220729945));
#114506=CARTESIAN_POINT('Ctrl Pts',(21.2599219862373,5.09680022375913,-7.81959377878623));
#114507=CARTESIAN_POINT('Ctrl Pts',(21.2531800695621,5.07365705542753,-7.6774836004288));
#114508=CARTESIAN_POINT('Ctrl Pts',(21.2464381528869,5.05654921504795,-7.53446510332613));
#114509=CARTESIAN_POINT('Ctrl Pts',(21.2396962362116,5.04551934956637,-7.39107767261309));
#114510=CARTESIAN_POINT('Ctrl Pts',(21.234587273223,5.03716101806669,-7.28241998492061));
#114511=CARTESIAN_POINT('Ctrl Pts',(21.2294783102344,5.03229187939357,-7.1735505847344));
#114512=CARTESIAN_POINT('Ctrl Pts',(21.2243693472458,5.03091055206464,-7.06470426108234));
#114513=CARTESIAN_POINT('Ctrl Pts',(21.2176540847332,5.02909492418669,-6.92163576783203));
#114514=CARTESIAN_POINT('Ctrl Pts',(21.2109388222206,5.03330382692002,-6.77836163457666));
#114515=CARTESIAN_POINT('Ctrl Pts',(21.204223559708,5.04355066274045,-6.63541758294017));
#114516=CARTESIAN_POINT('Ctrl Pts',(21.1975132922854,5.05378987654069,-6.4925798590002));
#114517=CARTESIAN_POINT('Ctrl Pts',(21.1908030248627,5.07005805418267,-6.35007209501922));
#114518=CARTESIAN_POINT('Ctrl Pts',(21.1840927574401,5.0923165571577,-6.20842943261171));
#114519=CARTESIAN_POINT('Ctrl Pts',(21.1773862402139,5.11456262042581,-6.06686593065854));
#114520=CARTESIAN_POINT('Ctrl Pts',(21.1706797229878,5.14279228431588,-5.92616693170634));
#114521=CARTESIAN_POINT('Ctrl Pts',(21.1639732057617,5.1769151576724,-5.78686176404052));
#114522=CARTESIAN_POINT('Ctrl Pts',(21.1572691966892,5.21102526950076,-5.64760869476631));
#114523=CARTESIAN_POINT('Ctrl Pts',(21.1505651876166,5.25102411227424,-5.50974877692657));
#114524=CARTESIAN_POINT('Ctrl Pts',(21.1438611785441,5.29677036811347,-5.3738003489467));
#114525=CARTESIAN_POINT('Ctrl Pts',(21.137157010186,5.34251771087248,-5.23784869086563));
#114526=CARTESIAN_POINT('Ctrl Pts',(21.1304528418279,5.39401263052893,-5.10380896672768));
#114527=CARTESIAN_POINT('Ctrl Pts',(21.1237486734698,5.45106410989234,-4.97218377998582));
#114528=CARTESIAN_POINT('Ctrl Pts',(21.1170447259729,5.50811370975889,-4.84056292948781));
#114529=CARTESIAN_POINT('Ctrl Pts',(21.1103407784761,5.57071935366059,-4.7113567955426));
#114530=CARTESIAN_POINT('Ctrl Pts',(21.1036368309793,5.63864230175156,-4.58504697062599));
#114531=CARTESIAN_POINT('Ctrl Pts',(21.0969291756063,5.7066028172431,-4.45866728519946));
#114532=CARTESIAN_POINT('Ctrl Pts',(21.0902215202333,5.77988633723191,-4.33518743528798));
#114533=CARTESIAN_POINT('Ctrl Pts',(21.0835138648603,5.85820842230719,-4.21506386817751));
#114534=CARTESIAN_POINT('Ctrl Pts',(21.0774380885725,5.92915235738501,-4.10625626252948));
#114535=CARTESIAN_POINT('Ctrl Pts',(21.0713623122848,6.00422960092619,-4.00020221885507));
#114536=CARTESIAN_POINT('Ctrl Pts',(21.065286535997,6.08319878352127,-3.89721939777838));
#114537=CARTESIAN_POINT('',(21.7216535043236,10.1294562983577,-12.0989999998127));
#114538=CARTESIAN_POINT('Ctrl Pts',(21.7216535043236,10.1294562983577,-12.0989999998127));
#114539=CARTESIAN_POINT('Ctrl Pts',(21.7145780823896,9.97829741836422,-12.0989987042859));
#114540=CARTESIAN_POINT('Ctrl Pts',(21.7075026604556,9.8271603213621,-12.092271455827));
#114541=CARTESIAN_POINT('Ctrl Pts',(21.7004272385216,9.67663880551781,-12.0788500409573));
#114542=CARTESIAN_POINT('Ctrl Pts',(21.6933497400828,9.52607311440785,-12.065424687152));
#114543=CARTESIAN_POINT('Ctrl Pts',(21.686272241644,9.37612366434497,-12.0453012699465));
#114544=CARTESIAN_POINT('Ctrl Pts',(21.6791947432053,9.22737926268248,-12.0185634573353));
#114545=CARTESIAN_POINT('Ctrl Pts',(21.6769530559598,9.18026679336472,-12.0100946722101));
#114546=CARTESIAN_POINT('Ctrl Pts',(21.6747113687143,9.13327515566229,-12.0009627140914));
#114547=CARTESIAN_POINT('Ctrl Pts',(21.6724696814689,9.08642286948864,-11.9911713154133));
#114548=CARTESIAN_POINT('Ctrl Pts',(21.6655384929631,8.94155786744673,-11.960896784428));
#114549=CARTESIAN_POINT('Ctrl Pts',(21.6586073044574,8.79798658804774,-11.9243058365266));
#114550=CARTESIAN_POINT('Ctrl Pts',(21.6516761159517,8.65626323121066,-11.8815340235511));
#114551=CARTESIAN_POINT('Ctrl Pts',(21.64474624141,8.51456674125142,-11.8387703189433));
#114552=CARTESIAN_POINT('Ctrl Pts',(21.6378163668684,8.37471779167141,-11.7898281825944));
#114553=CARTESIAN_POINT('Ctrl Pts',(21.6308864923267,8.2372559332038,-11.7348931763742));
#114554=CARTESIAN_POINT('Ctrl Pts',(21.6239563464653,8.09978869280394,-11.6799560193284));
#114555=CARTESIAN_POINT('Ctrl Pts',(21.6170262006039,7.9647090391401,-11.6190256426999));
#114556=CARTESIAN_POINT('Ctrl Pts',(21.6100960547425,7.83253754293167,-11.5523361552964));
#114557=CARTESIAN_POINT('Ctrl Pts',(21.6031662631196,7.70037280274875,-11.4856500767661));
#114558=CARTESIAN_POINT('Ctrl Pts',(21.5962364714968,7.57111621763294,-11.4132056266103));
#114559=CARTESIAN_POINT('Ctrl Pts',(21.5893066798739,7.44526470784607,-11.3352833697874));
#114560=CARTESIAN_POINT('Ctrl Pts',(21.5823752942246,7.31938424904482,-11.2573431888844));
#114561=CARTESIAN_POINT('Ctrl Pts',(21.5754439085753,7.19691071214243,-11.1739228579809));
#114562=CARTESIAN_POINT('Ctrl Pts',(21.568512522926,7.07831346210215,-11.0853471958881));
#114563=CARTESIAN_POINT('Ctrl Pts',(21.5643830274709,7.00765705517126,-11.0325766803587));
#114564=CARTESIAN_POINT('Ctrl Pts',(21.5602535320158,6.9383759408189,-10.9779771655619));
#114565=CARTESIAN_POINT('Ctrl Pts',(21.5561240365606,6.87056406102977,-10.9216243504048));
#114566=CARTESIAN_POINT('Ctrl Pts',(21.5491919803161,6.75673035668187,-10.8270266232852));
#114567=CARTESIAN_POINT('Ctrl Pts',(21.5422599240716,6.64699821171827,-10.7274524655712));
#114568=CARTESIAN_POINT('Ctrl Pts',(21.5353278678271,6.54179397638852,-10.6232811770744));
#114569=CARTESIAN_POINT('Ctrl Pts',(21.5283971552673,6.43661013346749,-10.5191300807637));
#114570=CARTESIAN_POINT('Ctrl Pts',(21.5214664427075,6.33595268411619,-10.4103838641845));
#114571=CARTESIAN_POINT('Ctrl Pts',(21.5145357301477,6.24021162379281,-10.297459162249));
#114572=CARTESIAN_POINT('Ctrl Pts',(21.5076047985457,6.14446753761436,-10.1845308913768));
#114573=CARTESIAN_POINT('Ctrl Pts',(21.5006738669437,6.05364036800616,-10.0674241210261));
#114574=CARTESIAN_POINT('Ctrl Pts',(21.4937429353417,5.96808061140313,-9.94658949842187));
#114575=CARTESIAN_POINT('Ctrl Pts',(21.4868123893406,5.88252561489794,-9.82576159842469));
#114576=CARTESIAN_POINT('Ctrl Pts',(21.4798818433394,5.80223763552051,-9.7012065317229));
#114577=CARTESIAN_POINT('Ctrl Pts',(21.4729512973382,5.72752452675666,-9.57340492984763));
#114578=CARTESIAN_POINT('Ctrl Pts',(21.4660192119694,5.65279482320388,-9.44557494151323));
#114579=CARTESIAN_POINT('Ctrl Pts',(21.4590871266005,5.58364263152974,-9.31449726290405));
#114580=CARTESIAN_POINT('Ctrl Pts',(21.4521550412316,5.5203307404732,-9.18067873310885));
#114581=CARTESIAN_POINT('Ctrl Pts',(21.4480294913719,5.48265140599206,-9.10103819387072));
#114582=CARTESIAN_POINT('Ctrl Pts',(21.4439039415122,5.44703976938654,-9.02042734711839));
#114583=CARTESIAN_POINT('Ctrl Pts',(21.4397783916525,5.41354327869334,-8.93895673050291));
#114584=CARTESIAN_POINT('Ctrl Pts',(21.4328288078177,5.35711766800913,-8.8017175988741));
#114585=CARTESIAN_POINT('Ctrl Pts',(21.425879223983,5.3066782204933,-8.66199295346232));
#114586=CARTESIAN_POINT('Ctrl Pts',(21.4189296401482,5.26242423305924,-8.52032051846249));
#114587=CARTESIAN_POINT('Ctrl Pts',(21.4119812825149,5.21817805390603,-8.37867308049059));
#114588=CARTESIAN_POINT('Ctrl Pts',(21.4050329248816,5.18011525469409,-8.23507885105442));
#114589=CARTESIAN_POINT('Ctrl Pts',(21.3980845672483,5.14838550186882,-8.09009144410335));
#114590=CARTESIAN_POINT('Ctrl Pts',(21.3911359899612,5.11665474599245,-7.94509945376403));
#114591=CARTESIAN_POINT('Ctrl Pts',(21.3841874126742,5.09125751019233,-7.79871451694216));
#114592=CARTESIAN_POINT('Ctrl Pts',(21.3772388353872,5.07229262147526,-7.6515017502624));
#114593=CARTESIAN_POINT('Ctrl Pts',(21.3702906875388,5.05332890483344,-7.50429808168186));
#114594=CARTESIAN_POINT('Ctrl Pts',(21.3633425396903,5.04079678109596,-7.35626701042103));
#114595=CARTESIAN_POINT('Ctrl Pts',(21.3563943918419,5.03474335699634,-7.20798016388597));
#114596=CARTESIAN_POINT('Ctrl Pts',(21.3494449282258,5.02868878656242,-7.05966523633523));
#114597=CARTESIAN_POINT('Ctrl Pts',(21.3424954646096,5.02911538076994,-6.91109476395886));
#114598=CARTESIAN_POINT('Ctrl Pts',(21.3355460009934,5.03601815715149,-6.76284242248547));
#114599=CARTESIAN_POINT('Ctrl Pts',(21.331508249577,5.04002878252507,-6.67670540028748));
#114600=CARTESIAN_POINT('Ctrl Pts',(21.3274704981606,5.04622466346145,-6.59067577933083));
#114601=CARTESIAN_POINT('Ctrl Pts',(21.3234327467442,5.0545967490254,-6.50486568161013));
#114602=CARTESIAN_POINT('Ctrl Pts',(21.31655060643,5.06886653971637,-6.35860676866734));
#114603=CARTESIAN_POINT('Ctrl Pts',(21.3096684661157,5.08946675265018,-6.21293115702204));
#114604=CARTESIAN_POINT('Ctrl Pts',(21.3027863258014,5.11632565505071,-6.06839708719742));
#114605=CARTESIAN_POINT('Ctrl Pts',(21.2959056901371,5.14317868525947,-5.92389461701757));
#114606=CARTESIAN_POINT('Ctrl Pts',(21.2890250544729,5.17628761360455,-5.78053352530322));
#114607=CARTESIAN_POINT('Ctrl Pts',(21.2821444188086,5.21552937377503,-5.63886309116306));
#114608=CARTESIAN_POINT('Ctrl Pts',(21.2752633519625,5.25477359306887,-5.49718377910633));
#114609=CARTESIAN_POINT('Ctrl Pts',(21.2683822851165,5.30015132574767,-5.35719566559861));
#114610=CARTESIAN_POINT('Ctrl Pts',(21.2615012182705,5.35148915214393,-5.21943454549694));
#114611=CARTESIAN_POINT('Ctrl Pts',(21.2546203142567,5.4028257636912,-5.08167668534937));
#114612=CARTESIAN_POINT('Ctrl Pts',(21.247739410243,5.46012206546334,-4.946146031246));
#114613=CARTESIAN_POINT('Ctrl Pts',(21.2408585062293,5.52315589001064,-4.81335989692717));
#114614=CARTESIAN_POINT('Ctrl Pts',(21.2339753023867,5.58621078257564,-4.68052938102991));
#114615=CARTESIAN_POINT('Ctrl Pts',(21.2270920985441,5.65500688289976,-4.55044552515016));
#114616=CARTESIAN_POINT('Ctrl Pts',(21.2202088947016,5.72927504815719,-4.42360302492416));
#114617=CARTESIAN_POINT('Ctrl Pts',(21.2158349637464,5.7764687437722,-4.34300097523082));
#114618=CARTESIAN_POINT('Ctrl Pts',(21.2114610327912,5.82587110691438,-4.26370729362511));
#114619=CARTESIAN_POINT('Ctrl Pts',(21.2070871018361,5.87740373338063,-4.1858432276432));
#114620=CARTESIAN_POINT('Ctrl Pts',(21.2015511092381,5.9426274969921,-4.08729231375261));
#114621=CARTESIAN_POINT('Ctrl Pts',(21.1960151166401,6.01128077510044,-3.99100686207785));
#114622=CARTESIAN_POINT('Ctrl Pts',(21.1904791240421,6.08319878352127,-3.89721939777839));
#114623=CARTESIAN_POINT('Ctrl Pts',(22.6904763725673,6.08319878352126,-3.8972193977784));
#114624=CARTESIAN_POINT('Ctrl Pts',(22.6832062449146,6.17769169863551,-3.77399225206862));
#114625=CARTESIAN_POINT('Ctrl Pts',(22.6759361172618,6.27782641665125,-3.65507385892176));
#114626=CARTESIAN_POINT('Ctrl Pts',(22.6686659896091,6.38318054496964,-3.54096956635808));
#114627=CARTESIAN_POINT('Ctrl Pts',(22.6617335873508,6.48364056877638,-3.4321658570933));
#114628=CARTESIAN_POINT('Ctrl Pts',(22.6548011850925,6.58884578356875,-3.32773933975731));
#114629=CARTESIAN_POINT('Ctrl Pts',(22.6478687828343,6.69839058953318,-3.22809209902919));
#114630=CARTESIAN_POINT('Ctrl Pts',(22.6409364801077,6.80793382271231,-3.12844628898247));
#114631=CARTESIAN_POINT('Ctrl Pts',(22.6340041773811,6.92181627608599,-3.03357983863798));
#114632=CARTESIAN_POINT('Ctrl Pts',(22.6270718746546,7.03959749637345,-2.94385607774054));
#114633=CARTESIAN_POINT('Ctrl Pts',(22.6201382212635,7.15740166472249,-2.85411483539414));
#114634=CARTESIAN_POINT('Ctrl Pts',(22.6132045678725,7.27910585338731,-2.76951848290543));
#114635=CARTESIAN_POINT('Ctrl Pts',(22.6062709144814,7.40423831077666,-2.69038868048967));
#114636=CARTESIAN_POINT('Ctrl Pts',(22.6052588898991,7.42250243731776,-2.67883902539102));
#114637=CARTESIAN_POINT('Ctrl Pts',(22.6042468653167,7.44083954937272,-2.66740575310795));
#114638=CARTESIAN_POINT('Ctrl Pts',(22.6032348407344,7.45924813015834,-2.65608978550349));
#114639=CARTESIAN_POINT('Ctrl Pts',(22.5963013558529,7.58536721737684,-2.57856292333584));
#114640=CARTESIAN_POINT('Ctrl Pts',(22.5893678709714,7.71488667542901,-2.50651889974946));
#114641=CARTESIAN_POINT('Ctrl Pts',(22.5824343860899,7.84731029346214,-2.44024001252559));
#114642=CARTESIAN_POINT('Ctrl Pts',(22.5755022191216,7.97970874048394,-2.37397372355758));
#114643=CARTESIAN_POINT('Ctrl Pts',(22.5685700521532,8.11500995065022,-2.31347053248643));
#114644=CARTESIAN_POINT('Ctrl Pts',(22.5616378851848,8.25269401104442,-2.25896632791746));
#114645=CARTESIAN_POINT('Ctrl Pts',(22.5547054748914,8.39038290426868,-2.20446021020359));
#114646=CARTESIAN_POINT('Ctrl Pts',(22.547773064598,8.53045450894211,-2.15595362514327));
#114647=CARTESIAN_POINT('Ctrl Pts',(22.5408406543045,8.6723693620486,-2.11363414141518));
#114648=CARTESIAN_POINT('Ctrl Pts',(22.5339086194588,8.81427652928531,-2.07131694963917));
#114649=CARTESIAN_POINT('Ctrl Pts',(22.526976584613,8.95802642811843,-2.03518628227907));
#114650=CARTESIAN_POINT('Ctrl Pts',(22.5200445497673,9.10306486807958,-2.00537970212354));
#114651=CARTESIAN_POINT('Ctrl Pts',(22.5131109730705,9.24813556807392,-1.97556649226857));
#114652=CARTESIAN_POINT('Ctrl Pts',(22.5061773963736,9.39449505792168,-1.95208024682281));
#114653=CARTESIAN_POINT('Ctrl Pts',(22.4992438196768,9.54157877108382,-1.93500744042109));
#114654=CARTESIAN_POINT('Ctrl Pts',(22.4951256117266,9.62893935615773,-1.92486702226029));
#114655=CARTESIAN_POINT('Ctrl Pts',(22.4910074037764,9.71655526433281,-1.91698814636579));
#114656=CARTESIAN_POINT('Ctrl Pts',(22.4868891958262,9.80430724843803,-1.9113802780782));
#114657=CARTESIAN_POINT('Ctrl Pts',(22.4799556232921,9.95204984768639,-1.90193865638155));
#114658=CARTESIAN_POINT('Ctrl Pts',(22.4730220507579,10.1002293919555,-1.89893406231333));
#114659=CARTESIAN_POINT('Ctrl Pts',(22.4660884782238,10.2482752299219,-1.90238355260451));
#114660=CARTESIAN_POINT('Ctrl Pts',(22.4591562219442,10.3962929631829,-1.90583238805183));
#114661=CARTESIAN_POINT('Ctrl Pts',(22.4522239656647,10.5441767104752,-1.91573285564485));
#114662=CARTESIAN_POINT('Ctrl Pts',(22.4452917093852,10.6913566113617,-1.93204990669116));
#114663=CARTESIAN_POINT('Ctrl Pts',(22.4383592081633,10.838541712659,-1.94836753427928));
#114664=CARTESIAN_POINT('Ctrl Pts',(22.4314267069415,10.9850225888615,-1.9711021658943));
#114665=CARTESIAN_POINT('Ctrl Pts',(22.4244942057197,11.1302347335151,-2.00016690347203));
#114666=CARTESIAN_POINT('Ctrl Pts',(22.4175620792479,11.2754390284404,-2.02923006989818));
#114667=CARTESIAN_POINT('Ctrl Pts',(22.410629952776,11.4193744050801,-2.06462259177438));
#114668=CARTESIAN_POINT('Ctrl Pts',(22.4036978263042,11.5614867616133,-2.10620649040397));
#114669=CARTESIAN_POINT('Ctrl Pts',(22.3967641577058,11.7036307325799,-2.14779963982234));
#114670=CARTESIAN_POINT('Ctrl Pts',(22.3898304891073,11.8439505557084,-2.19558682522712));
#114671=CARTESIAN_POINT('Ctrl Pts',(22.3828968205088,11.9819068852309,-2.24938006871217));
#114672=CARTESIAN_POINT('Ctrl Pts',(22.3787790639786,12.063836179762,-2.28132671809408));
#114673=CARTESIAN_POINT('Ctrl Pts',(22.3746613074483,12.1449322010469,-2.31539070984882));
#114674=CARTESIAN_POINT('Ctrl Pts',(22.370543550918,12.2250851901569,-2.35152458210273));
#114675=CARTESIAN_POINT('Ctrl Pts',(22.3636099924989,12.3600483499194,-2.41236749798139));
#114676=CARTESIAN_POINT('Ctrl Pts',(22.3566764340798,12.4923832519696,-2.47910262136328));
#114677=CARTESIAN_POINT('Ctrl Pts',(22.3497428756607,12.6215776949439,-2.55147780017193));
#114678=CARTESIAN_POINT('Ctrl Pts',(22.3428106341768,12.7507475991896,-2.62383923229903));
#114679=CARTESIAN_POINT('Ctrl Pts',(22.3358783926929,12.8767779461898,-2.7018384210654));
#114680=CARTESIAN_POINT('Ctrl Pts',(22.328946151209,12.9991816332476,-2.78517754539985));
#114681=CARTESIAN_POINT('Ctrl Pts',(22.3220136656563,13.1215896298659,-2.86851960391878));
#114682=CARTESIAN_POINT('Ctrl Pts',(22.3150811801037,13.2403704359038,-2.95720179093612));
#114683=CARTESIAN_POINT('Ctrl Pts',(22.308148694551,13.3550659593708,-3.0508829794816));
#114684=CARTESIAN_POINT('Ctrl Pts',(22.3012165842048,13.4697552751808,-3.14455909772731));
#114685=CARTESIAN_POINT('Ctrl Pts',(22.2942844738585,13.580359495408,-3.24323346626158));
#114686=CARTESIAN_POINT('Ctrl Pts',(22.2873523635122,13.6864536413925,-3.34652469654105));
#114687=CARTESIAN_POINT('Ctrl Pts',(22.2804187116004,13.7925713806377,-3.44983889676766));
#114688=CARTESIAN_POINT('Ctrl Pts',(22.2734850596885,13.8941768046595,-3.55777177953251));
#114689=CARTESIAN_POINT('Ctrl Pts',(22.2665514077766,13.9908813866036,-3.66990468797189));
#114690=CARTESIAN_POINT('Ctrl Pts',(22.2624335738543,14.0483133738203,-3.73649942045101));
#114691=CARTESIAN_POINT('Ctrl Pts',(22.2583157399321,14.1040175187899,-3.80457484120395));
#114692=CARTESIAN_POINT('Ctrl Pts',(22.2541979060098,14.1579190618731,-3.874037610281));
#114693=CARTESIAN_POINT('Ctrl Pts',(22.2472642956059,14.248678501657,-3.99099904861213));
#114694=CARTESIAN_POINT('Ctrl Pts',(22.240330685202,14.3343563570106,-4.11193599116586));
#114695=CARTESIAN_POINT('Ctrl Pts',(22.2333970747981,14.4146181346602,-4.23638577728254));
#114696=CARTESIAN_POINT('Ctrl Pts',(22.2264647807023,14.4948646750486,-4.36081193728546));
#114697=CARTESIAN_POINT('Ctrl Pts',(22.2195324866065,14.569697010104,-4.48874933264206));
#114698=CARTESIAN_POINT('Ctrl Pts',(22.2126001925108,14.6388242094336,-4.61970670416093));
#114699=CARTESIAN_POINT('Ctrl Pts',(22.2056676539223,14.7079538467869,-4.75066869437094));
#114700=CARTESIAN_POINT('Ctrl Pts',(22.1987351153338,14.7713777885139,-4.88465058310104));
#114701=CARTESIAN_POINT('Ctrl Pts',(22.1918025767453,14.8288510170149,-5.0211364324741));
#114702=CARTESIAN_POINT('Ctrl Pts',(22.1848704132515,14.8863211358465,-5.1576148970895));
#114703=CARTESIAN_POINT('Ctrl Pts',(22.1779382497577,14.9378410582831,-5.29659674622179));
#114704=CARTESIAN_POINT('Ctrl Pts',(22.1710060862639,14.9832138788456,-5.43754597433969));
#114705=CARTESIAN_POINT('Ctrl Pts',(22.1640723815,15.028596787423,-5.57852654055607));
#114706=CARTESIAN_POINT('Ctrl Pts',(22.1571386767362,15.0678297619024,-5.72147504499835));
#114707=CARTESIAN_POINT('Ctrl Pts',(22.1502049719723,15.1007655570025,-5.86583962255727));
#114708=CARTESIAN_POINT('Ctrl Pts',(22.1460874016821,15.1203244300737,-5.95157031282543));
#114709=CARTESIAN_POINT('Ctrl Pts',(22.1419698313918,15.1376635206223,-6.03780011735071));
#114710=CARTESIAN_POINT('Ctrl Pts',(22.1378522611016,15.1527604864707,-6.12441157781638));
#114711=CARTESIAN_POINT('Ctrl Pts',(22.1309189472056,15.1781813040225,-6.27025108997362));
#114712=CARTESIAN_POINT('Ctrl Pts',(22.1239856333095,15.1972510326479,-6.41722360612244));
#114713=CARTESIAN_POINT('Ctrl Pts',(22.1170523194135,15.2098907721861,-6.56476374015239));
#114714=CARTESIAN_POINT('Ctrl Pts',(22.1101203233419,15.2225281092719,-6.71227583102913));
#114715=CARTESIAN_POINT('Ctrl Pts',(22.1031883272702,15.2287378674464,-6.86035499529274));
#114716=CARTESIAN_POINT('Ctrl Pts',(22.0962563311985,15.2284930298674,-7.00843097644238));
#114717=CARTESIAN_POINT('Ctrl Pts',(22.089324090006,15.2282481836307,-7.1565121936757));
#114718=CARTESIAN_POINT('Ctrl Pts',(22.0823918488135,15.2215482821266,-7.30458989694499));
#114719=CARTESIAN_POINT('Ctrl Pts',(22.075459607621,15.2084184326879,-7.45209352362448));
#114720=CARTESIAN_POINT('Ctrl Pts',(22.0685277404533,15.195289291662,-7.59958919183699));
#114721=CARTESIAN_POINT('Ctrl Pts',(22.0615958732855,15.1757309271479,-7.7465105161877));
#114722=CARTESIAN_POINT('Ctrl Pts',(22.0546640061178,15.1498203546765,-7.89229173279893));
#114723=CARTESIAN_POINT('Ctrl Pts',(22.0477305934374,15.1239040052452,-8.038105452445));
#114724=CARTESIAN_POINT('Ctrl Pts',(22.040797180757,15.0916326758373,-8.18277823079126));
#114725=CARTESIAN_POINT('Ctrl Pts',(22.0338637680765,15.0531346874517,-8.32575354592097));
#114726=CARTESIAN_POINT('Ctrl Pts',(22.0297447174488,15.030263531423,-8.41069332791254));
#114727=CARTESIAN_POINT('Ctrl Pts',(22.0256256668211,15.0051957146653,-8.49503421516273));
#114728=CARTESIAN_POINT('Ctrl Pts',(22.0215066161934,14.9779665423999,-8.57866183434858));
#114729=CARTESIAN_POINT('Ctrl Pts',(22.0145723805751,14.9321274612027,-8.71944515265239));
#114730=CARTESIAN_POINT('Ctrl Pts',(22.0076381449568,14.8801445592657,-8.85825478409665));
#114731=CARTESIAN_POINT('Ctrl Pts',(22.0007039093386,14.8222129650008,-8.99455409255137));
#114732=CARTESIAN_POINT('Ctrl Pts',(21.9937709880668,14.7642923513531,-9.13082756621661));
#114733=CARTESIAN_POINT('Ctrl Pts',(21.986838066795,14.7004254241925,-9.26459136227122));
#114734=CARTESIAN_POINT('Ctrl Pts',(21.9799051455232,14.6308554344628,-9.39532884018717));
#114735=CARTESIAN_POINT('Ctrl Pts',(21.9729719829147,14.5612830229847,-9.52607086910665));
#114736=CARTESIAN_POINT('Ctrl Pts',(21.9660388203062,14.4860073039592,-9.65378607580445));
#114737=CARTESIAN_POINT('Ctrl Pts',(21.9591056576977,14.4053177264321,-9.77798196004382));
#114738=CARTESIAN_POINT('Ctrl Pts',(21.9521728734695,14.3246325525718,-9.9021710662419));
#114739=CARTESIAN_POINT('Ctrl Pts',(21.9452400892412,14.23853429223,-10.0228409576983));
#114740=CARTESIAN_POINT('Ctrl Pts',(21.9383073050129,14.1473560123797,-10.1395276816401));
#114741=CARTESIAN_POINT('Ctrl Pts',(21.9313729900041,14.0561576000789,-10.2562401703768));
#114742=CARTESIAN_POINT('Ctrl Pts',(21.9244386749953,13.9598771305219,-10.3689674737665));
#114743=CARTESIAN_POINT('Ctrl Pts',(21.9175043599865,13.8588886754882,-10.4772778300189));
#114744=CARTESIAN_POINT('Ctrl Pts',(21.9133898970861,13.7989673637105,-10.541543578253));
#114745=CARTESIAN_POINT('Ctrl Pts',(21.9092754341856,13.7373893106772,-10.6042549247956));
#114746=CARTESIAN_POINT('Ctrl Pts',(21.9051609712852,13.6742389692849,-10.6653276305991));
#114747=CARTESIAN_POINT('Ctrl Pts',(21.8982288511239,13.5678421526517,-10.7682240098965));
#114748=CARTESIAN_POINT('Ctrl Pts',(21.8912967309625,13.4569435049872,-10.8665024520393));
#114749=CARTESIAN_POINT('Ctrl Pts',(21.8843646108012,13.3419664401948,-10.959780343734));
#114750=CARTESIAN_POINT('Ctrl Pts',(21.877433811209,13.2270112785383,-11.0530404659862));
#114751=CARTESIAN_POINT('Ctrl Pts',(21.8705030116169,13.1079795066484,-11.1413017300309));
#114752=CARTESIAN_POINT('Ctrl Pts',(21.8635722120248,12.9853276996924,-11.2242217211777));
#114753=CARTESIAN_POINT('Ctrl Pts',(21.8566411598445,12.8626714227769,-11.3071447342857));
#114754=CARTESIAN_POINT('Ctrl Pts',(21.8497101076642,12.7363951190217,-11.3847258969099));
#114755=CARTESIAN_POINT('Ctrl Pts',(21.8427790554839,12.6069848824144,-11.4566657556304));
#114756=CARTESIAN_POINT('Ctrl Pts',(21.8358483702673,12.4775814974173,-11.5286018055031));
#114757=CARTESIAN_POINT('Ctrl Pts',(21.8289176850508,12.3450448012554,-11.5948969892324));
#114758=CARTESIAN_POINT('Ctrl Pts',(21.8219869998343,12.209886058069,-11.6552975038543));
#114759=CARTESIAN_POINT('Ctrl Pts',(21.8150547479171,12.0746967618724,-11.7157116721808));
#114760=CARTESIAN_POINT('Ctrl Pts',(21.8081224959999,11.9368845365068,-11.7702283738593));
#114761=CARTESIAN_POINT('Ctrl Pts',(21.8011902440826,11.796981800889,-11.81864145208));
#114762=CARTESIAN_POINT('Ctrl Pts',(21.7970652715141,11.7137339683553,-11.8474492077709));
#114763=CARTESIAN_POINT('Ctrl Pts',(21.7929402989456,11.6297463168939,-11.8740967543871));
#114764=CARTESIAN_POINT('Ctrl Pts',(21.788815326377,11.5451338329821,-11.8985489536103));
#114765=CARTESIAN_POINT('Ctrl Pts',(21.781841763805,11.4020903481749,-11.939887153677));
#114766=CARTESIAN_POINT('Ctrl Pts',(21.7748682012329,11.2572131443299,-11.9749619273583));
#114767=CARTESIAN_POINT('Ctrl Pts',(21.7678946386609,11.1110621236963,-12.0036323603283));
#114768=CARTESIAN_POINT('Ctrl Pts',(21.7609226052006,10.9649431499895,-12.0322965066555));
#114769=CARTESIAN_POINT('Ctrl Pts',(21.7539505717403,10.8175512332713,-12.0545590528571));
#114770=CARTESIAN_POINT('Ctrl Pts',(21.7469785382801,10.669456698842,-12.0703301434301));
#114771=CARTESIAN_POINT('Ctrl Pts',(21.7400073493926,10.5213801041739,-12.0860993235369));
#114772=CARTESIAN_POINT('Ctrl Pts',(21.7330361605051,10.3726013821705,-12.0953785825651));
#114773=CARTESIAN_POINT('Ctrl Pts',(21.7260649716176,10.2236966737367,-12.0981298518826));
#114774=CARTESIAN_POINT('Ctrl Pts',(21.7245944825346,10.192287002918,-12.0987101993042));
#114775=CARTESIAN_POINT('Ctrl Pts',(21.7231239934515,10.1608717378449,-12.0990002690569));
#114776=CARTESIAN_POINT('Ctrl Pts',(21.7216535043684,10.1294562993151,-12.0989999998127));
#114777=CARTESIAN_POINT('Origin',(-26.8463464956315,10.1295,-7.));
#114778=CARTESIAN_POINT('',(-21.5963464956315,10.1291161856969,-12.0989999855547));
#114779=CARTESIAN_POINT('Ctrl Pts',(-22.5651720736884,14.1754919335065,
-3.89745664672419));
#114780=CARTESIAN_POINT('Ctrl Pts',(-22.5448385295376,13.9111214980616,
-3.55278411761959));
#114781=CARTESIAN_POINT('Ctrl Pts',(-22.4857231037507,13.0157743410226,
-2.64786717956705));
#114782=CARTESIAN_POINT('Ctrl Pts',(-22.3878257963277,11.0466612589386,
-1.77459151989547));
#114783=CARTESIAN_POINT('Ctrl Pts',(-22.2714801514196,8.49288304070303,
-1.95345842253097));
#114784=CARTESIAN_POINT('Ctrl Pts',(-22.1551345065114,6.32026199879215,
-3.30737376532056));
#114785=CARTESIAN_POINT('Ctrl Pts',(-22.0387888616032,5.03442895202576,
-5.52111017618096));
#114786=CARTESIAN_POINT('Ctrl Pts',(-21.922443216695,4.93530635993922,-8.0791637580032));
#114787=CARTESIAN_POINT('Ctrl Pts',(-21.8060975717868,6.0448778396091,-10.3860101436405));
#114788=CARTESIAN_POINT('Ctrl Pts',(-21.6973986661372,7.9715431412064,-11.8045112188381));
#114789=CARTESIAN_POINT('Ctrl Pts',(-21.6274816421238,9.46413915462446,
-12.0984964029847));
#114790=CARTESIAN_POINT('Ctrl Pts',(-21.5963464997463,10.1291160878984,
-12.0991317151048));
#114791=CARTESIAN_POINT('Ctrl Pts',(-21.5963464956315,10.1291161856969,
-12.0989999855547));
#114792=CARTESIAN_POINT('Ctrl Pts',(-21.5886997577445,10.2924291785527,
-12.0990122785264));
#114793=CARTESIAN_POINT('Ctrl Pts',(-21.5810530198574,10.4557419617455,
-12.0911739196201));
#114794=CARTESIAN_POINT('Ctrl Pts',(-21.5734062819704,10.6183440341081,
-12.0755130292727));
#114795=CARTESIAN_POINT('Ctrl Pts',(-21.5666848517297,10.761270142277,-12.0617472138972));
#114796=CARTESIAN_POINT('Ctrl Pts',(-21.5599634214889,10.9036700321504,
-12.0419345290273));
#114797=CARTESIAN_POINT('Ctrl Pts',(-21.5532419912482,11.0450086188271,
-12.0161384519223));
#114798=CARTESIAN_POINT('Ctrl Pts',(-21.5465222109883,11.1863125096208,
-11.9903487072541));
#114799=CARTESIAN_POINT('Ctrl Pts',(-21.5398024307283,11.3265552547391,
-11.9585785632498));
#114800=CARTESIAN_POINT('Ctrl Pts',(-21.5330826504684,11.4652102525116,
-11.9209429097822));
#114801=CARTESIAN_POINT('Ctrl Pts',(-21.5263615518046,11.6038924540449,
-11.8832998722942));
#114802=CARTESIAN_POINT('Ctrl Pts',(-21.5196404531407,11.7409859290593,
-11.8397891166586));
#114803=CARTESIAN_POINT('Ctrl Pts',(-21.5129193544769,11.8759772620419,
-11.7905759750964));
#114804=CARTESIAN_POINT('Ctrl Pts',(-21.5061977698631,12.0109783551886,
-11.7413592753181));
#114805=CARTESIAN_POINT('Ctrl Pts',(-21.4994761852493,12.1438766594992,
-11.6864394991817));
#114806=CARTESIAN_POINT('Ctrl Pts',(-21.4927546006356,12.2741773917404,
-11.6260306835729));
#114807=CARTESIAN_POINT('Ctrl Pts',(-21.4860285543178,12.4045646159827,
-11.5655817693456));
#114808=CARTESIAN_POINT('Ctrl Pts',(-21.479302508,12.5323504905475,-11.4996366941743));
#114809=CARTESIAN_POINT('Ctrl Pts',(-21.4725764616822,12.6570630553875,
-11.4284563903284));
#114810=CARTESIAN_POINT('Ctrl Pts',(-21.4674045201422,12.7529598221028,
-11.3737228436212));
#114811=CARTESIAN_POINT('Ctrl Pts',(-21.4622325786022,12.8470398696579,
-11.3158948186789));
#114812=CARTESIAN_POINT('Ctrl Pts',(-21.4570606370622,12.9390999696984,
-11.255108577965));
#114813=CARTESIAN_POINT('Ctrl Pts',(-21.4497817937609,13.0686627339555,
-11.1695597530969));
#114814=CARTESIAN_POINT('Ctrl Pts',(-21.4425029504596,13.1943036068353,
-11.0780978347688));
#114815=CARTESIAN_POINT('Ctrl Pts',(-21.4352241071583,13.3155153827349,
-10.9810936915597));
#114816=CARTESIAN_POINT('Ctrl Pts',(-21.427946142148,13.4367125327922,-10.8841012532143));
#114817=CARTESIAN_POINT('Ctrl Pts',(-21.4206681771377,13.553481456089,-10.7815680846603));
#114818=CARTESIAN_POINT('Ctrl Pts',(-21.4133902121274,13.6653475008962,
-10.6739057487102));
#114819=CARTESIAN_POINT('Ctrl Pts',(-21.4061165971437,13.7771466835695,
-10.5663077623448));
#114820=CARTESIAN_POINT('Ctrl Pts',(-21.39884298216,13.884048659969,-10.4535869088841));
#114821=CARTESIAN_POINT('Ctrl Pts',(-21.3915693671764,13.9856148483401,
-10.3361923320473));
#114822=CARTESIAN_POINT('Ctrl Pts',(-21.3843006041387,14.0871132858521,
-10.2188760645726));
#114823=CARTESIAN_POINT('Ctrl Pts',(-21.377031841101,14.1832828744343,-10.0968924881681));
#114824=CARTESIAN_POINT('Ctrl Pts',(-21.3697630780634,14.2737238199281,
-9.97072548889001));
#114825=CARTESIAN_POINT('Ctrl Pts',(-21.362503319337,14.3640527300697,-9.8447147812575));
#114826=CARTESIAN_POINT('Ctrl Pts',(-21.3552435606107,14.4486670178919,
-9.714531202894));
#114827=CARTESIAN_POINT('Ctrl Pts',(-21.3479838018843,14.5272087473904,
-9.58068959255577));
#114828=CARTESIAN_POINT('Ctrl Pts',(-21.3455608653075,14.5534219641621,
-9.53602010071664));
#114829=CARTESIAN_POINT('Ctrl Pts',(-21.3431379287308,14.5789591128104,
-9.49094340429971));
#114830=CARTESIAN_POINT('Ctrl Pts',(-21.340714992154,14.6038079371955,-9.44547939740844));
#114831=CARTESIAN_POINT('Ctrl Pts',(-21.3339843753385,14.6728348844358,
-9.31918603413384));
#114832=CARTESIAN_POINT('Ctrl Pts',(-21.3272537585231,14.7365235713096,
-9.18994468860557));
#114833=CARTESIAN_POINT('Ctrl Pts',(-21.3205231417076,14.7946316255852,
-9.05823903275719));
#114834=CARTESIAN_POINT('Ctrl Pts',(-21.3137927443259,14.852737785403,-8.92653767081938));
#114835=CARTESIAN_POINT('Ctrl Pts',(-21.3070623469442,14.9052635284585,
-8.79237249361583));
#114836=CARTESIAN_POINT('Ctrl Pts',(-21.3003319495625,14.9520141566811,
-8.65624823278712));
#114837=CARTESIAN_POINT('Ctrl Pts',(-21.2935981100412,14.9987886946639,
-8.52005435367601));
#114838=CARTESIAN_POINT('Ctrl Pts',(-21.28686427052,15.0397820953059,-8.38189973457362));
#114839=CARTESIAN_POINT('Ctrl Pts',(-21.2801304309987,15.0748490349447,
-8.24230588929287));
#114840=CARTESIAN_POINT('Ctrl Pts',(-21.2733949256715,15.1099246493843,
-8.10267751152055));
#114841=CARTESIAN_POINT('Ctrl Pts',(-21.2666594203442,15.1390707988718,
-7.96160955465916));
#114842=CARTESIAN_POINT('Ctrl Pts',(-21.259923915017,15.1621931252,-7.8196346183301));
#114843=CARTESIAN_POINT('Ctrl Pts',(-21.2531821581971,15.1853369122869,
-7.67752790936666));
#114844=CARTESIAN_POINT('Ctrl Pts',(-21.2464404013771,15.2024456529537,
-7.53451290148324));
#114845=CARTESIAN_POINT('Ctrl Pts',(-21.2396986445572,15.2134767052047,
-7.39112895691341));
#114846=CARTESIAN_POINT('Ctrl Pts',(-21.2345888787867,15.2218374477692,
-7.28245426104888));
#114847=CARTESIAN_POINT('Ctrl Pts',(-21.2294791130163,15.2267078994303,
-7.17356777436203));
#114848=CARTESIAN_POINT('Ctrl Pts',(-21.2243693472458,15.2280894461353,
-7.06470440292566));
#114849=CARTESIAN_POINT('Ctrl Pts',(-21.2176540790633,15.229905078602,-6.92163586176665));
#114850=CARTESIAN_POINT('Ctrl Pts',(-21.2109388108808,15.2256961764928,
-6.77836167525376));
#114851=CARTESIAN_POINT('Ctrl Pts',(-21.2042235426983,15.2154493359987,
-6.63541756535092));
#114852=CARTESIAN_POINT('Ctrl Pts',(-21.1975132699025,15.2052101179746,
-6.49257978941473));
#114853=CARTESIAN_POINT('Ctrl Pts',(-21.1908029971066,15.1889419313426,
-6.3500719684068));
#114854=CARTESIAN_POINT('Ctrl Pts',(-21.1840927243108,15.1666834132725,
-6.2084292444435));
#114855=CARTESIAN_POINT('Ctrl Pts',(-21.1773862020136,15.14443733591,-6.06686568728304));
#114856=CARTESIAN_POINT('Ctrl Pts',(-21.1706796797165,15.116207652359,-5.92616662852227));
#114857=CARTESIAN_POINT('Ctrl Pts',(-21.1639731574193,15.0820847524494,
-5.78686139711654));
#114858=CARTESIAN_POINT('Ctrl Pts',(-21.1572691435834,15.0479746156336,
-5.64760827047765));
#114859=CARTESIAN_POINT('Ctrl Pts',(-21.1505651297475,15.0079757415206,
-5.50974829121759));
#114860=CARTESIAN_POINT('Ctrl Pts',(-21.1438611159116,14.9622294466977,
-5.37379979860372));
#114861=CARTESIAN_POINT('Ctrl Pts',(-21.1371569432884,14.916482068355,-5.23784808599431));
#114862=CARTESIAN_POINT('Ctrl Pts',(-21.1304527706652,14.864987106323,-5.10380830382993));
#114863=CARTESIAN_POINT('Ctrl Pts',(-21.123748598042,14.8079355765373,-4.97218305653825));
#114864=CARTESIAN_POINT('Ctrl Pts',(-21.1170446465545,14.7508859285836,
-4.84056215087628));
#114865=CARTESIAN_POINT('Ctrl Pts',(-21.1103406950669,14.6882802290009,
-4.71135595904673));
#114866=CARTESIAN_POINT('Ctrl Pts',(-21.1036367435794,14.6203572164572,
-4.58504607468499));
#114867=CARTESIAN_POINT('Ctrl Pts',(-21.096929084689,14.5523966412952,-4.45866633873984));
#114868=CARTESIAN_POINT('Ctrl Pts',(-21.0902214257986,14.479113053607,-4.3351864363366));
#114869=CARTESIAN_POINT('Ctrl Pts',(-21.0835137669082,14.4007908917012,
-4.21506281606388));
#114870=CARTESIAN_POINT('Ctrl Pts',(-21.0774380110089,14.3298471622981,
-4.10625558444275));
#114871=CARTESIAN_POINT('Ctrl Pts',(-21.0713622551095,14.2547701490326,
-4.00020189286647));
#114872=CARTESIAN_POINT('Ctrl Pts',(-21.0652864992102,14.1758012177496,
-3.89721939943571));
#114873=CARTESIAN_POINT('',(-21.7216535043236,10.1295436686122,-12.098999999813));
#114874=CARTESIAN_POINT('Ctrl Pts',(-21.7216535043236,10.1295436686122,
-12.098999999813));
#114875=CARTESIAN_POINT('Ctrl Pts',(-21.7145780772905,10.2807026533976,
-12.0989987052645));
#114876=CARTESIAN_POINT('Ctrl Pts',(-21.7075026502575,10.4318398568485,
-12.0922714484638));
#114877=CARTESIAN_POINT('Ctrl Pts',(-21.7004272232244,10.582361479932,-12.0788500155049));
#114878=CARTESIAN_POINT('Ctrl Pts',(-21.693349719895,10.7329272738466,-12.0654246440032));
#114879=CARTESIAN_POINT('Ctrl Pts',(-21.6862722165656,10.8828768275428,
-12.0453011997449));
#114880=CARTESIAN_POINT('Ctrl Pts',(-21.6791947132363,11.0316213327613,
-12.0185633503003));
#114881=CARTESIAN_POINT('Ctrl Pts',(-21.6769530359805,11.0787335923755,
-12.0100945971002));
#114882=CARTESIAN_POINT('Ctrl Pts',(-21.6747113587247,11.1257250216099,
-12.0009626767532));
#114883=CARTESIAN_POINT('Ctrl Pts',(-21.6724696814689,11.1725771008058,
-11.9911713216213));
#114884=CARTESIAN_POINT('Ctrl Pts',(-21.665538500834,11.3174419439415,-11.9608968247447));
#114885=CARTESIAN_POINT('Ctrl Pts',(-21.6586073201992,11.4610130681156,
-11.9243059246399));
#114886=CARTESIAN_POINT('Ctrl Pts',(-21.6516761395644,11.6027362745548,
-11.88153417271));
#114887=CARTESIAN_POINT('Ctrl Pts',(-21.6447462728878,11.7444326142333,
-11.8387705291094));
#114888=CARTESIAN_POINT('Ctrl Pts',(-21.6378164062113,11.884281418354,-11.7898284670043));
#114889=CARTESIAN_POINT('Ctrl Pts',(-21.6308865395347,12.0217431373186,
-11.7348935478288));
#114890=CARTESIAN_POINT('Ctrl Pts',(-21.6239564014542,12.1592102398846,
-11.6799564771618));
#114891=CARTESIAN_POINT('Ctrl Pts',(-21.6170262633738,12.2942897616118,
-11.6190261995686));
#114892=CARTESIAN_POINT('Ctrl Pts',(-21.6100961252933,12.426461132908,-11.5523368234249));
#114893=CARTESIAN_POINT('Ctrl Pts',(-21.6031663413856,12.5586257494336,
-11.4856508555187));
#114894=CARTESIAN_POINT('Ctrl Pts',(-21.5962365574778,12.6878822178597,
-11.4132065281025));
#114895=CARTESIAN_POINT('Ctrl Pts',(-21.5893067735701,12.8137336190688,
-11.3352844056949));
#114896=CARTESIAN_POINT('Ctrl Pts',(-21.5823753954677,12.9396139723548,
-11.2573443573264));
#114897=CARTESIAN_POINT('Ctrl Pts',(-21.5754440173652,13.0620874116896,
-11.1739241703709));
#114898=CARTESIAN_POINT('Ctrl Pts',(-21.5685126392628,13.1806845732687,
-11.0853486631923));
#114899=CARTESIAN_POINT('Ctrl Pts',(-21.5643831050287,13.2513416679423,
-11.0325776869467));
#114900=CARTESIAN_POINT('Ctrl Pts',(-21.5602535707947,13.3206234444385,
-10.9779776769825));
#114901=CARTESIAN_POINT('Ctrl Pts',(-21.5561240365606,13.3884359580966,
-10.9216243345105));
#114902=CARTESIAN_POINT('Ctrl Pts',(-21.5491919873467,13.5022695420679,
-10.8270267064872));
#114903=CARTESIAN_POINT('Ctrl Pts',(-21.5422599381329,13.6120015769791,
-10.7274526569437));
#114904=CARTESIAN_POINT('Ctrl Pts',(-21.535327888919,13.7172057131023,-10.6232814845348));
#114905=CARTESIAN_POINT('Ctrl Pts',(-21.5283971834842,13.8223894553827,
-10.5191305057286));
#114906=CARTESIAN_POINT('Ctrl Pts',(-21.5214664780495,13.9230468150587,
-10.4103844146959));
#114907=CARTESIAN_POINT('Ctrl Pts',(-21.5145357726147,14.0187877971565,
-10.2974598452277));
#114908=CARTESIAN_POINT('Ctrl Pts',(-21.5076048482097,14.1145318041177,
-10.1845317079939));
#114909=CARTESIAN_POINT('Ctrl Pts',(-21.5006739238046,14.2053589060595,
-10.06742507829));
#114910=CARTESIAN_POINT('Ctrl Pts',(-21.4937429993995,14.2909186070078,
-9.94659060224677));
#114911=CARTESIAN_POINT('Ctrl Pts',(-21.4868124606186,14.3764735475678,
-9.82576284921712));
#114912=CARTESIAN_POINT('Ctrl Pts',(-21.4798819218377,14.4567614830456,
-9.70120793542299));
#114913=CARTESIAN_POINT('Ctrl Pts',(-21.4729513830568,14.5314745604009,
-9.57340649132294));
#114914=CARTESIAN_POINT('Ctrl Pts',(-21.4660193048808,14.6062042328509,
-9.44557666026405));
#114915=CARTESIAN_POINT('Ctrl Pts',(-21.4590872267048,14.6753564058714,
-9.31449914377409));
#114916=CARTESIAN_POINT('Ctrl Pts',(-21.4521551485288,14.7386682911608,
-9.18068077988451));
#114917=CARTESIAN_POINT('Ctrl Pts',(-21.4480295629033,14.7763479879615,
-9.10103956631653));
#114918=CARTESIAN_POINT('Ctrl Pts',(-21.4439039772779,14.8119599512988,
-9.020428027734));
#114919=CARTESIAN_POINT('Ctrl Pts',(-21.4397783916524,14.8454567318764,
-8.93895670479501));
#114920=CARTESIAN_POINT('Ctrl Pts',(-21.4328287564197,14.9018827590196,
-8.80171655812195));
#114921=CARTESIAN_POINT('Ctrl Pts',(-21.425879121187,14.9523225305843,-8.661990870534));
#114922=CARTESIAN_POINT('Ctrl Pts',(-21.4189294859543,14.9965767489365,
-8.52031737474841));
#114923=CARTESIAN_POINT('Ctrl Pts',(-21.4119810766083,15.0408231610291,
-8.37866886957668));
#114924=CARTESIAN_POINT('Ctrl Pts',(-21.4050326672623,15.0788860995113,
-8.23507355414718));
#114925=CARTESIAN_POINT('Ctrl Pts',(-21.3980842579163,15.110615897284,-8.09008505072978));
#114926=CARTESIAN_POINT('Ctrl Pts',(-21.3911356289697,15.1423466978592,
-7.94509196503175));
#114927=CARTESIAN_POINT('Ctrl Pts',(-21.3841870000231,15.1677438841323,
-7.79870592238976));
#114928=CARTESIAN_POINT('Ctrl Pts',(-21.3772383710765,15.1867086284737,
-7.65149204760402));
#114929=CARTESIAN_POINT('Ctrl Pts',(-21.3702901717336,15.2056722003069,
-7.50428727441542));
#114930=CARTESIAN_POINT('Ctrl Pts',(-21.3633419723906,15.2182040846995,
-7.35625509628934));
#114931=CARTESIAN_POINT('Ctrl Pts',(-21.3563937730477,15.2242571742947,
-7.20796714878315));
#114932=CARTESIAN_POINT('Ctrl Pts',(-21.349444258653,15.2303114095286,-7.05965113554095));
#114933=CARTESIAN_POINT('Ctrl Pts',(-21.3424947442583,15.2298843862783,
-6.91107958341258));
#114934=CARTESIAN_POINT('Ctrl Pts',(-21.3355452298636,15.2229810863828,
-6.76282617627361));
#114935=CARTESIAN_POINT('Ctrl Pts',(-21.3315077354905,15.2189704414799,
-6.67669464777756));
#114936=CARTESIAN_POINT('Ctrl Pts',(-21.3274702411173,15.2127748193448,
-6.59067051003166));
#114937=CARTESIAN_POINT('Ctrl Pts',(-21.3234327467442,15.204403268655,-6.50486586282613));
#114938=CARTESIAN_POINT('Ctrl Pts',(-21.3165507415352,15.190133761349,-6.35860980041302));
#114939=CARTESIAN_POINT('Ctrl Pts',(-21.3096687363261,15.1695340759322,
-6.2129369909791));
#114940=CARTESIAN_POINT('Ctrl Pts',(-21.3027867311171,15.1426759370888,
-6.06840565491519));
#114941=CARTESIAN_POINT('Ctrl Pts',(-21.2959062311046,15.1158236725188,
-5.92390592999837));
#114942=CARTESIAN_POINT('Ctrl Pts',(-21.2890257310922,15.0827157467963,
-5.78054751496072));
#114943=CARTESIAN_POINT('Ctrl Pts',(-21.2821452310798,15.043475218225,-5.63887966929049));
#114944=CARTESIAN_POINT('Ctrl Pts',(-21.2752642995611,15.0042322287083,
-5.49720293900956));
#114945=CARTESIAN_POINT('Ctrl Pts',(-21.2683833680424,14.9588559542226,
-5.35721731924835));
#114946=CARTESIAN_POINT('Ctrl Pts',(-21.2615024365237,14.9075198065233,
-5.21945858557822));
#114947=CARTESIAN_POINT('Ctrl Pts',(-21.2546216674167,14.8561848705188,
-5.08170310344812));
#114948=CARTESIAN_POINT('Ctrl Pts',(-21.2477408983096,14.7988904640697,
-4.94617472034563));
#114949=CARTESIAN_POINT('Ctrl Pts',(-21.2408601292026,14.7358587467217,
-4.81339073072018));
#114950=CARTESIAN_POINT('Ctrl Pts',(-21.2339770585298,14.672805945736,-4.68056232584397));
#114951=CARTESIAN_POINT('Ctrl Pts',(-21.227093987857,14.6040121460503,-4.5504804560366));
#114952=CARTESIAN_POINT('Ctrl Pts',(-21.2202109171841,14.52974648257,-4.4236397975768));
#114953=CARTESIAN_POINT('Ctrl Pts',(-21.2158363120681,14.4825461897285,
-4.34302493543258));
#114954=CARTESIAN_POINT('Ctrl Pts',(-21.2114617069521,14.433136544005,-4.2637188372088));
#114955=CARTESIAN_POINT('Ctrl Pts',(-21.2070871018361,14.3815959889042,
-4.1858428080249));
#114956=CARTESIAN_POINT('Ctrl Pts',(-21.2015511135273,14.3163722937598,
-4.08729201871722));
#114957=CARTESIAN_POINT('Ctrl Pts',(-21.1960151252186,14.2477191097718,
-3.99100671202062));
#114958=CARTESIAN_POINT('Ctrl Pts',(-21.1904791369099,14.1758012177496,
-3.89721939943572));
#114959=CARTESIAN_POINT('Ctrl Pts',(-22.6904763727661,14.1758012177496,
-3.89721939943571));
#114960=CARTESIAN_POINT('Ctrl Pts',(-22.6832062450968,14.0813083024994,
-3.77399225344413));
#114961=CARTESIAN_POINT('Ctrl Pts',(-22.6759361174275,13.9811735843942,
-3.6550738601199));
#114962=CARTESIAN_POINT('Ctrl Pts',(-22.6686659897582,13.8758194560258,
-3.54096956743624));
#114963=CARTESIAN_POINT('Ctrl Pts',(-22.6617335870542,13.7753594259407,
-3.43216585130876));
#114964=CARTESIAN_POINT('Ctrl Pts',(-22.6548011843501,13.6701542043166,
-3.32773932770549));
#114965=CARTESIAN_POINT('Ctrl Pts',(-22.6478687816461,13.5606093910262,
-3.22809208134504));
#114966=CARTESIAN_POINT('Ctrl Pts',(-22.6409364784718,13.4510661504903,
-3.12844626563806));
#114967=CARTESIAN_POINT('Ctrl Pts',(-22.6340041752975,13.3371836892631,
-3.03357981027087));
#114968=CARTESIAN_POINT('Ctrl Pts',(-22.6270718721233,13.2194024606833,
-2.94385604502711));
#114969=CARTESIAN_POINT('Ctrl Pts',(-22.6201382182847,13.101598284045,-2.85411479833708));
#114970=CARTESIAN_POINT('Ctrl Pts',(-22.6132045644461,12.9798940866522,
-2.7695184421809));
#114971=CARTESIAN_POINT('Ctrl Pts',(-22.6062709106076,12.8547616201541,
-2.69038863681246));
#114972=CARTESIAN_POINT('Ctrl Pts',(-22.6052588873165,12.8364975167663,
-2.67883899676501));
#114973=CARTESIAN_POINT('Ctrl Pts',(-22.6042468640255,12.8181604280522,
-2.66740573923635));
#114974=CARTESIAN_POINT('Ctrl Pts',(-22.6032348407344,12.7997518707891,
-2.65608978608592));
#114975=CARTESIAN_POINT('Ctrl Pts',(-22.5963013561296,12.6736327888376,
-2.57856292711801));
#114976=CARTESIAN_POINT('Ctrl Pts',(-22.5893678715248,12.5441133362429,
-2.50651890621843));
#114977=CARTESIAN_POINT('Ctrl Pts',(-22.5824343869199,12.4116897238054,
-2.4402400211681));
#114978=CARTESIAN_POINT('Ctrl Pts',(-22.5755022202333,12.2792912824762,
-2.37397373442229));
#114979=CARTESIAN_POINT('Ctrl Pts',(-22.5685700535467,12.1439900781449,
-2.31347054505179));
#114980=CARTESIAN_POINT('Ctrl Pts',(-22.5616378868601,12.0063060236781,
-2.25896634166286));
#114981=CARTESIAN_POINT('Ctrl Pts',(-22.5547054768533,11.8686171364782,
-2.20446022516737));
#114982=CARTESIAN_POINT('Ctrl Pts',(-22.5477730668465,11.7285455379248,
-2.15595364079637));
#114983=CARTESIAN_POINT('Ctrl Pts',(-22.5408406568397,11.5866306909856,
-2.11363415723017));
#114984=CARTESIAN_POINT('Ctrl Pts',(-22.5339086222827,11.4447235299589,
-2.07131696562884));
#114985=CARTESIAN_POINT('Ctrl Pts',(-22.5269765877257,11.3009736373842,
-2.03518629791231));
#114986=CARTESIAN_POINT('Ctrl Pts',(-22.5200445531686,11.155935203683,-2.00537971687135));
#114987=CARTESIAN_POINT('Ctrl Pts',(-22.5131109767612,11.0108645099633,
-1.97556650613346));
#114988=CARTESIAN_POINT('Ctrl Pts',(-22.5061774003538,10.8645050263921,
-1.9520802592744));
#114989=CARTESIAN_POINT('Ctrl Pts',(-22.4992438239464,10.7174213194626,
-1.93500745093131));
#114990=CARTESIAN_POINT('Ctrl Pts',(-22.495125614573,10.6300607042532,-1.92486702768973));
#114991=CARTESIAN_POINT('Ctrl Pts',(-22.4910074051996,10.5424447657293,
-1.91698814828052));
#114992=CARTESIAN_POINT('Ctrl Pts',(-22.4868891958262,10.4546927511912,
-1.9113802780545));
#114993=CARTESIAN_POINT('Ctrl Pts',(-22.4799556232166,10.3069501501543,
-1.90193865625436));
#114994=CARTESIAN_POINT('Ctrl Pts',(-22.4730220506069,10.158770604134,-1.89893406224141));
#114995=CARTESIAN_POINT('Ctrl Pts',(-22.4660884779973,10.0107247644674,
-1.90238355273524));
#114996=CARTESIAN_POINT('Ctrl Pts',(-22.4591562216396,9.86270702945001,
-1.90583238838649));
#114997=CARTESIAN_POINT('Ctrl Pts',(-22.4522239652819,9.71482328045241,
-1.91573285633567));
#114998=CARTESIAN_POINT('Ctrl Pts',(-22.4452917089242,9.56764337792384,
-1.93204990787901));
#114999=CARTESIAN_POINT('Ctrl Pts',(-22.4383592076211,9.420458274917,-1.94836753597166));
#115000=CARTESIAN_POINT('Ctrl Pts',(-22.4314267063179,9.27397739706878,
-1.97110216823797));
#115001=CARTESIAN_POINT('Ctrl Pts',(-22.4244942050148,9.12876525084503,
-2.00016690660241));
#115002=CARTESIAN_POINT('Ctrl Pts',(-22.41756207846,8.98356095431581,-2.02923007382199));
#115003=CARTESIAN_POINT('Ctrl Pts',(-22.4106299519053,8.83962557614821,
-2.06462259662998));
#115004=CARTESIAN_POINT('Ctrl Pts',(-22.4036978253505,8.69751321817358,
-2.10620649631859));
#115005=CARTESIAN_POINT('Ctrl Pts',(-22.3967641566674,8.55536924572963,
-2.14779964680663));
#115006=CARTESIAN_POINT('Ctrl Pts',(-22.3898304879842,8.41504942121115,
-2.19558683341147));
#115007=CARTESIAN_POINT('Ctrl Pts',(-22.3828968193011,8.27709309039585,
-2.24938007821602));
#115008=CARTESIAN_POINT('Ctrl Pts',(-22.3787790631734,8.19516380410787,
-2.28132672486794));
#115009=CARTESIAN_POINT('Ctrl Pts',(-22.3746613070457,8.11406779091711,
-2.31539071346896));
#115010=CARTESIAN_POINT('Ctrl Pts',(-22.370543550918,8.03391480971792,-2.35152458215918));
#115011=CARTESIAN_POINT('Ctrl Pts',(-22.3636099925257,7.89895165060084,
-2.41236749775123));
#115012=CARTESIAN_POINT('Ctrl Pts',(-22.3566764341333,7.76661674914673,
-2.47910262080128));
#115013=CARTESIAN_POINT('Ctrl Pts',(-22.3497428757409,7.63742230671767,
-2.55147779924112));
#115014=CARTESIAN_POINT('Ctrl Pts',(-22.3428106342854,7.5082524030468,-2.62383923098281));
#115015=CARTESIAN_POINT('Ctrl Pts',(-22.3358783928298,7.3822220565691,-2.70183841932422));
#115016=CARTESIAN_POINT('Ctrl Pts',(-22.3289461513742,7.25981836998035,
-2.78517754320212));
#115017=CARTESIAN_POINT('Ctrl Pts',(-22.322013665852,7.13741037386829,-2.86851960123916));
#115018=CARTESIAN_POINT('Ctrl Pts',(-22.3150811803298,7.01862956828097,
-2.95720178773977));
#115019=CARTESIAN_POINT('Ctrl Pts',(-22.3081486948075,6.90393404520842,
-3.05088297574135));
#115020=CARTESIAN_POINT('Ctrl Pts',(-22.3012165844928,6.78924472981139,
-3.14455909342806));
#115021=CARTESIAN_POINT('Ctrl Pts',(-22.2942844741781,6.67864050993959,
-3.24323346137456));
#115022=CARTESIAN_POINT('Ctrl Pts',(-22.2873523638634,6.5725463642529,-3.34652469104477));
#115023=CARTESIAN_POINT('Ctrl Pts',(-22.2804187119845,6.4664286253275,-3.44983889064064));
#115024=CARTESIAN_POINT('Ctrl Pts',(-22.2734850601056,6.36482320156598,
-3.55777177275135));
#115025=CARTESIAN_POINT('Ctrl Pts',(-22.2665514082267,6.2681186198229,-3.66990468052016));
#115026=CARTESIAN_POINT('Ctrl Pts',(-22.2624335741544,6.21068663035953,
-3.73649941534445));
#115027=CARTESIAN_POINT('Ctrl Pts',(-22.2583157400821,6.15498248326484,
-3.80457483855878));
#115028=CARTESIAN_POINT('Ctrl Pts',(-22.2541979060098,6.10108093818732,
-3.87403761020318));
#115029=CARTESIAN_POINT('Ctrl Pts',(-22.247264295271,6.01032149396891,-3.99099905424433));
#115030=CARTESIAN_POINT('Ctrl Pts',(-22.2403306845322,5.92464363472474,
-4.11193600283431));
#115031=CARTESIAN_POINT('Ctrl Pts',(-22.2333970737934,5.84438185374589,
-4.23638579525945));
#115032=CARTESIAN_POINT('Ctrl Pts',(-22.2264647793601,5.76413530999738,
-4.36081196161838));
#115033=CARTESIAN_POINT('Ctrl Pts',(-22.2195324849268,5.68930297214713,
-4.48874936360589));
#115034=CARTESIAN_POINT('Ctrl Pts',(-22.2126001904935,5.62017577060433,
-4.61970674197797));
#115035=CARTESIAN_POINT('Ctrl Pts',(-22.2056676515668,5.55104613103073,
-4.75066873905461));
#115036=CARTESIAN_POINT('Ctrl Pts',(-22.1987351126401,5.48762218766616,
-4.88465063487431));
#115037=CARTESIAN_POINT('Ctrl Pts',(-22.1918025737133,5.43014895812622,
-5.02113649150837));
#115038=CARTESIAN_POINT('Ctrl Pts',(-22.1848704098817,5.37267883825905,
-5.15761496337642));
#115039=CARTESIAN_POINT('Ctrl Pts',(-22.1779382460501,5.3211589153847,-5.2965968199325));
#115040=CARTESIAN_POINT('Ctrl Pts',(-22.1710060822185,5.27578609499789,
-5.43754605559421));
#115041=CARTESIAN_POINT('Ctrl Pts',(-22.1640723771204,5.23040318662025,
-5.57852662928132));
#115042=CARTESIAN_POINT('Ctrl Pts',(-22.1571386720224,5.19117021294783,
-5.72147514131237));
#115043=CARTESIAN_POINT('Ctrl Pts',(-22.1502049669243,5.15823441927751,
-5.8658397265272));
#115044=CARTESIAN_POINT('Ctrl Pts',(-22.1460873983168,5.13867555599091,
-5.95157038217522));
#115045=CARTESIAN_POINT('Ctrl Pts',(-22.1419698297092,5.12133647341795,
-6.03780015164788));
#115046=CARTESIAN_POINT('Ctrl Pts',(-22.1378522611016,5.10623951371014,
-6.12441157677879));
#115047=CARTESIAN_POINT('Ctrl Pts',(-22.1309189485113,5.08081870089726,
-6.27025106157069));
#115048=CARTESIAN_POINT('Ctrl Pts',(-22.123985635921,5.06174897458694,-6.41722355017293));
#115049=CARTESIAN_POINT('Ctrl Pts',(-22.1170523233307,5.04910923496427,
-6.56476365668796));
#115050=CARTESIAN_POINT('Ctrl Pts',(-22.1101203285711,5.03647189780609,
-6.71227571991427));
#115051=CARTESIAN_POINT('Ctrl Pts',(-22.1031883338116,5.03026213714831,
-6.86035485655776));
#115052=CARTESIAN_POINT('Ctrl Pts',(-22.096256339052,5.03050696985794,-7.00843081032554));
#115053=CARTESIAN_POINT('Ctrl Pts',(-22.0893240991684,5.03075181122517,
-7.15651200024495));
#115054=CARTESIAN_POINT('Ctrl Pts',(-22.0823918592848,5.03745170547963,
-7.30458967643834));
#115055=CARTESIAN_POINT('Ctrl Pts',(-22.0754596194012,5.05058154531326,
-7.45209327648446));
#115056=CARTESIAN_POINT('Ctrl Pts',(-22.0685277535374,5.0637106767437,-7.5995889181684));
#115057=CARTESIAN_POINT('Ctrl Pts',(-22.0615958876737,5.08326902931621,
-7.74651021643196));
#115058=CARTESIAN_POINT('Ctrl Pts',(-22.0546640218099,5.10917958752434,
-7.89229140760191));
#115059=CARTESIAN_POINT('Ctrl Pts',(-22.0477306104145,5.13509592276128,
-8.03810510220675));
#115060=CARTESIAN_POINT('Ctrl Pts',(-22.0407971990191,5.16736723568739,
-8.18277785615135));
#115061=CARTESIAN_POINT('Ctrl Pts',(-22.0338637876236,5.20586520532844,
-8.32575314772379));
#115062=CARTESIAN_POINT('Ctrl Pts',(-22.0297447304802,5.22873639063859,
-8.41069306582378));
#115063=CARTESIAN_POINT('Ctrl Pts',(-22.0256256733368,5.25380424364472,
-8.49503408736322));
#115064=CARTESIAN_POINT('Ctrl Pts',(-22.0215066161934,5.28103345893842,
-8.57866183845887));
#115065=CARTESIAN_POINT('Ctrl Pts',(-22.0145723772777,5.32687256185952,
-8.71944522307671));
#115066=CARTESIAN_POINT('Ctrl Pts',(-22.0076381383619,5.37885549112866,
-8.85825491842587));
#115067=CARTESIAN_POINT('Ctrl Pts',(-22.0007038994462,5.43678711804054,
-8.99455428792793));
#115068=CARTESIAN_POINT('Ctrl Pts',(-21.993770974864,5.49470776444206,-9.1308278228951));
#115069=CARTESIAN_POINT('Ctrl Pts',(-21.9868380502819,5.55857472969261,
-9.26459167738601));
#115070=CARTESIAN_POINT('Ctrl Pts',(-21.9799051256997,5.62814476255884,
-9.39532921043455));
#115071=CARTESIAN_POINT('Ctrl Pts',(-21.9729719597937,5.69771721704527,
-9.52607129424495));
#115072=CARTESIAN_POINT('Ctrl Pts',(-21.9660387938876,5.77299298410511,
-9.65378655254162));
#115073=CARTESIAN_POINT('Ctrl Pts',(-21.9591056279816,5.85368261440674,
-9.77798248465653));
#115074=CARTESIAN_POINT('Ctrl Pts',(-21.9521728404709,5.93436784086443,
-9.90217163845925));
#115075=CARTESIAN_POINT('Ctrl Pts',(-21.9452400529602,6.02046615852026,
-10.0228415738131));
#115076=CARTESIAN_POINT('Ctrl Pts',(-21.9383072654495,6.11164450011518,
-10.1395283375127));
#115077=CARTESIAN_POINT('Ctrl Pts',(-21.9313729472104,6.20284297347965,
-10.2562408651272));
#115078=CARTESIAN_POINT('Ctrl Pts',(-21.9244386289712,6.29912350845597,
-10.3689682033144));
#115079=CARTESIAN_POINT('Ctrl Pts',(-21.9175043107321,6.40011203297749,
-10.4772785898498));
#115080=CARTESIAN_POINT('Ctrl Pts',(-21.9133898642498,6.4600331189647,-10.5415440696718));
#115081=CARTESIAN_POINT('Ctrl Pts',(-21.9092754177675,6.5216109328709,-10.6042551600696));
#115082=CARTESIAN_POINT('Ctrl Pts',(-21.9051609712852,6.58476102287579,
-10.6653276230177));
#115083=CARTESIAN_POINT('Ctrl Pts',(-21.8982288574645,6.69115774320861,
-10.7682239096234));
#115084=CARTESIAN_POINT('Ctrl Pts',(-21.8912967436438,6.80205628720019,
-10.8665022681371));
#115085=CARTESIAN_POINT('Ctrl Pts',(-21.8843646298231,6.91703324183498,
-10.959780085773));
#115086=CARTESIAN_POINT('Ctrl Pts',(-21.8774338365917,7.0319882930012,-11.0530401336937));
#115087=CARTESIAN_POINT('Ctrl Pts',(-21.8705030433603,7.15101994789269,
-11.1413013330034));
#115088=CARTESIAN_POINT('Ctrl Pts',(-21.863572250129,7.27367163221487,-11.2242212695068));
#115089=CARTESIAN_POINT('Ctrl Pts',(-21.8566412042781,7.39632778705076,
-11.3071442283471));
#115090=CARTESIAN_POINT('Ctrl Pts',(-21.8497101584272,7.52260396312254,
-11.3847253467466));
#115091=CARTESIAN_POINT('Ctrl Pts',(-21.8427791125763,7.65201406730398,
-11.4566651717729));
#115092=CARTESIAN_POINT('Ctrl Pts',(-21.8358484336565,7.78141732048679,
-11.5286011882895));
#115093=CARTESIAN_POINT('Ctrl Pts',(-21.8289177547367,7.91395388012075,
-11.5948963491388));
#115094=CARTESIAN_POINT('Ctrl Pts',(-21.8219870758168,8.04911248293015,
-11.6552968518474));
#115095=CARTESIAN_POINT('Ctrl Pts',(-21.8150548300911,8.18430164079854,
-11.7157110091875));
#115096=CARTESIAN_POINT('Ctrl Pts',(-21.8081225843653,8.32211372406473,
-11.7702277106694));
#115097=CARTESIAN_POINT('Ctrl Pts',(-21.8011903386395,8.46201631468121,
-11.8186407999762));
#115098=CARTESIAN_POINT('Ctrl Pts',(-21.797065334552,8.54526477138227,-11.8474488081137));
#115099=CARTESIAN_POINT('Ctrl Pts',(-21.7929403304645,8.62925305861412,
-11.8740965742915));
#115100=CARTESIAN_POINT('Ctrl Pts',(-21.788815326377,8.71386618713863,-11.898548959425));
#115101=CARTESIAN_POINT('Ctrl Pts',(-21.7818417513357,8.85690992448683,
-11.939887231837));
#115102=CARTESIAN_POINT('Ctrl Pts',(-21.7748681762943,9.00178738562049,
-11.9749620552806));
#115103=CARTESIAN_POINT('Ctrl Pts',(-21.7678946012529,9.14793866626696,
-12.0036325152953));
#115104=CARTESIAN_POINT('Ctrl Pts',(-21.7609225553009,9.29405790045778,
-12.0322966887649));
#115105=CARTESIAN_POINT('Ctrl Pts',(-21.7539505093488,9.44145008039454,
-12.0545592393556));
#115106=CARTESIAN_POINT('Ctrl Pts',(-21.7469784633968,9.58954487878361,
-12.0703303114365));
#115107=CARTESIAN_POINT('Ctrl Pts',(-21.740007262077,9.73762173614916,-12.0860994729225));
#115108=CARTESIAN_POINT('Ctrl Pts',(-21.7330360607571,9.88640072158192,
-12.0953786905622));
#115109=CARTESIAN_POINT('Ctrl Pts',(-21.7260648594373,10.0353056921974,
-12.0981298955968));
#115110=CARTESIAN_POINT('Ctrl Pts',(-21.7245944077477,10.0667145635801,
-12.0987102136662));
#115111=CARTESIAN_POINT('Ctrl Pts',(-21.723123956058,10.0981290288572,-12.0990002688469));
#115112=CARTESIAN_POINT('Ctrl Pts',(-21.7216535043684,10.1295436676547,
-12.098999999813));
#115113=CARTESIAN_POINT('Origin',(11.,-13.5,-22.));
#115114=CARTESIAN_POINT('',(7.,-13.5,-22.));
#115115=CARTESIAN_POINT('Origin',(11.,-13.5,-22.));
#115116=CARTESIAN_POINT('',(7.,-13.5,-16.));
#115117=CARTESIAN_POINT('',(7.,-13.5,-22.));
#115118=CARTESIAN_POINT('Origin',(11.,-13.5,-16.));
#115119=CARTESIAN_POINT('Origin',(2.22044604925031E-15,2.25,-16.));
#115120=CARTESIAN_POINT('Origin',(11.,17.5,-22.));
#115121=CARTESIAN_POINT('',(6.55407155365721,16.8045,-22.));
#115122=CARTESIAN_POINT('',(9.25758668237251,21.6489752747581,-22.));
#115123=CARTESIAN_POINT('Origin',(11.,17.5,-22.));
#115124=CARTESIAN_POINT('',(6.55407155365721,16.8045,-16.));
#115125=CARTESIAN_POINT('',(6.55407155365721,16.8045,-22.));
#115126=CARTESIAN_POINT('',(9.25758668237251,21.6489752747581,-16.));
#115127=CARTESIAN_POINT('Origin',(11.,17.5,-16.));
#115128=CARTESIAN_POINT('',(9.25758668237251,21.6489752747581,-22.));
#115129=CARTESIAN_POINT('Origin',(2.22044604925031E-15,2.25,-16.));
#115130=CARTESIAN_POINT('',(9.25758668237251,21.5062266006623,-16.));
#115131=CARTESIAN_POINT('',(9.25758668237251,11.8781133003311,-16.));
#115132=CARTESIAN_POINT('',(7.0995,16.8045,-16.));
#115133=CARTESIAN_POINT('',(-3.54975,16.8045,-16.));
#115134=CARTESIAN_POINT('',(7.0995,19.4175,-16.));
#115135=CARTESIAN_POINT('',(7.0995,9.52725,-16.));
#115136=CARTESIAN_POINT('Origin',(10.7505,17.8045,-16.));
#115137=CARTESIAN_POINT('Origin',(-11.,-13.5,-22.));
#115138=CARTESIAN_POINT('',(-15.,-13.5,-22.));
#115139=CARTESIAN_POINT('Origin',(-11.,-13.5,-22.));
#115140=CARTESIAN_POINT('',(-15.,-13.5,-16.));
#115141=CARTESIAN_POINT('',(-15.,-13.5,-22.));
#115142=CARTESIAN_POINT('Origin',(-11.,-13.5,-16.));
#115143=CARTESIAN_POINT('Origin',(2.22044604925031E-15,2.25,-16.));
#115144=CARTESIAN_POINT('Origin',(-11.,17.5,-22.));
#115145=CARTESIAN_POINT('',(-9.25758668237251,21.6489752747581,-22.));
#115146=CARTESIAN_POINT('',(-6.55407155365721,16.8045,-22.));
#115147=CARTESIAN_POINT('Origin',(-11.,17.5,-22.));
#115148=CARTESIAN_POINT('',(-9.25758668237251,21.6489752747581,-16.));
#115149=CARTESIAN_POINT('',(-9.25758668237251,21.6489752747581,-22.));
#115150=CARTESIAN_POINT('',(-6.55407155365721,16.8045,-16.));
#115151=CARTESIAN_POINT('Origin',(-11.,17.5,-16.));
#115152=CARTESIAN_POINT('',(-6.55407155365721,16.8045,-22.));
#115153=CARTESIAN_POINT('Origin',(2.22044604925031E-15,2.25,-16.));
#115154=CARTESIAN_POINT('',(-7.0995,16.8045,-16.));
#115155=CARTESIAN_POINT('',(-7.0995,19.4175,-16.));
#115156=CARTESIAN_POINT('',(-7.0995,10.83375,-16.));
#115157=CARTESIAN_POINT('',(-3.54975,16.8045,-16.));
#115158=CARTESIAN_POINT('',(-9.25758668237251,21.5062266006622,-16.));
#115159=CARTESIAN_POINT('',(-9.25758668237251,13.2726133003311,-16.));
#115160=CARTESIAN_POINT('Origin',(-10.7505,17.8045,-16.));
#115161=CARTESIAN_POINT('Origin',(1.5089639216641E-15,6.00000008940697,
-22.));
#115162=CARTESIAN_POINT('',(-5.,6.00000008940697,-22.));
#115163=CARTESIAN_POINT('Origin',(1.5089639216641E-15,6.00000008940697,
-22.));
#115164=CARTESIAN_POINT('',(-5.,6.00000008940697,-16.));
#115165=CARTESIAN_POINT('',(-5.,6.00000008940697,-22.));
#115166=CARTESIAN_POINT('Origin',(1.5089639216641E-15,6.00000008940697,
-16.));
#115167=CARTESIAN_POINT('Origin',(2.22044604925031E-15,2.25,-16.));
#115168=CARTESIAN_POINT('Origin',(7.0995,16.8045,0.));
#115169=CARTESIAN_POINT('',(7.0995,16.8045,0.));
#115170=CARTESIAN_POINT('',(7.0995,16.8045,0.));
#115171=CARTESIAN_POINT('',(7.0995,19.4175,0.));
#115172=CARTESIAN_POINT('',(7.0995,16.8045,0.));
#115173=CARTESIAN_POINT('',(7.0995,19.4175,0.));
#115174=CARTESIAN_POINT('Origin',(-9.25758668237251,24.2952266006623,0.));
#115175=CARTESIAN_POINT('',(-9.25758668237251,24.2952266006623,-22.));
#115176=CARTESIAN_POINT('',(-9.25758668237251,21.5062266006623,-22.));
#115177=CARTESIAN_POINT('',(-9.25758668237251,24.2952266006623,0.));
#115178=CARTESIAN_POINT('',(-9.25758668237251,24.2952266006623,0.));
#115179=CARTESIAN_POINT('',(-9.25758668237251,21.5062266006623,0.));
#115180=CARTESIAN_POINT('',(-9.25758668237251,21.5062266006623,0.));
#115181=CARTESIAN_POINT('',(-9.25758668237251,21.5062266006623,0.));
#115182=CARTESIAN_POINT('Origin',(-7.0995,16.8045,0.));
#115183=CARTESIAN_POINT('',(7.0995,16.8045,-22.));
#115184=CARTESIAN_POINT('',(-7.0995,16.8045,0.));
#115185=CARTESIAN_POINT('',(-7.0995,16.8045,0.));
#115186=CARTESIAN_POINT('',(7.0995,16.8045,0.));
#115187=CARTESIAN_POINT('Origin',(0.,1.05261330033112,-22.));
#115188=CARTESIAN_POINT('',(9.25758668237251,24.2952266006623,-22.));
#115189=CARTESIAN_POINT('',(9.25758668237251,21.5062266006623,-22.));
#115190=CARTESIAN_POINT('',(9.06658668237251,24.4862266006622,-22.));
#115191=CARTESIAN_POINT('Origin',(9.06658668237251,24.2952266006623,-22.));
#115192=CARTESIAN_POINT('',(7.30158668237251,24.4862266006622,-22.));
#115193=CARTESIAN_POINT('',(9.06658668237251,24.4862266006622,-22.));
#115194=CARTESIAN_POINT('',(7.11058668237251,24.6772266006623,-22.));
#115195=CARTESIAN_POINT('Origin',(7.30158668237251,24.6772266006623,-22.));
#115196=CARTESIAN_POINT('',(7.11058668237251,25.8032266006622,-22.));
#115197=CARTESIAN_POINT('',(7.11058668237251,24.6772266006623,-22.));
#115198=CARTESIAN_POINT('',(7.36458668237251,26.0572266006622,-22.));
#115199=CARTESIAN_POINT('Origin',(7.36458668237251,25.8032266006622,-22.));
#115200=CARTESIAN_POINT('',(18.734,24.211,-22.));
#115201=CARTESIAN_POINT('',(7.36458668237251,26.0572266006622,-22.));
#115202=CARTESIAN_POINT('',(23.734,19.211,-22.));
#115203=CARTESIAN_POINT('Origin',(18.734,19.211,-22.));
#115204=CARTESIAN_POINT('',(23.734,6.1295,-22.));
#115205=CARTESIAN_POINT('',(23.734,19.211,-22.));
#115206=CARTESIAN_POINT('',(23.534,6.1295,-22.));
#115207=CARTESIAN_POINT('',(11.867,6.1295,-22.));
#115208=CARTESIAN_POINT('',(23.534,-5.8705,-22.));
#115209=CARTESIAN_POINT('',(23.534,0.591056650165565,-22.));
#115210=CARTESIAN_POINT('',(23.734,-5.8705,-22.));
#115211=CARTESIAN_POINT('',(11.867,-5.8705,-22.));
#115212=CARTESIAN_POINT('',(23.734,-18.952,-22.));
#115213=CARTESIAN_POINT('',(23.734,19.211,-22.));
#115214=CARTESIAN_POINT('',(18.734,-23.952,-22.));
#115215=CARTESIAN_POINT('Origin',(18.734,-18.952,-22.));
#115216=CARTESIAN_POINT('',(-18.734,-23.952,-22.));
#115217=CARTESIAN_POINT('',(-18.734,-23.952,-22.));
#115218=CARTESIAN_POINT('',(-23.734,-18.952,-22.));
#115219=CARTESIAN_POINT('Origin',(-18.734,-18.952,-22.));
#115220=CARTESIAN_POINT('',(-23.734,-5.8705,-22.));
#115221=CARTESIAN_POINT('',(-23.734,19.211,-22.));
#115222=CARTESIAN_POINT('',(-23.534,-5.8705,-22.));
#115223=CARTESIAN_POINT('',(-11.867,-5.8705,-22.));
#115224=CARTESIAN_POINT('',(-23.534,6.1295,-22.));
#115225=CARTESIAN_POINT('',(-23.534,0.591056650165565,-22.));
#115226=CARTESIAN_POINT('',(-23.734,6.1295,-22.));
#115227=CARTESIAN_POINT('',(-11.867,6.1295,-22.));
#115228=CARTESIAN_POINT('',(-23.734,19.211,-22.));
#115229=CARTESIAN_POINT('',(-23.734,19.211,-22.));
#115230=CARTESIAN_POINT('',(-18.734,24.211,-22.));
#115231=CARTESIAN_POINT('Origin',(-18.734,19.211,-22.));
#115232=CARTESIAN_POINT('',(-7.36458668237251,26.0572266006623,-22.));
#115233=CARTESIAN_POINT('',(-7.36458668237251,26.0572266006622,-22.));
#115234=CARTESIAN_POINT('',(-7.11058668237251,25.8032266006623,-22.));
#115235=CARTESIAN_POINT('Origin',(-7.36458668237251,25.8032266006623,-22.));
#115236=CARTESIAN_POINT('',(-7.11058668237251,24.6772266006623,-22.));
#115237=CARTESIAN_POINT('',(-7.11058668237251,24.6772266006623,-22.));
#115238=CARTESIAN_POINT('',(-7.30158668237251,24.4862266006622,-22.));
#115239=CARTESIAN_POINT('Origin',(-7.30158668237251,24.6772266006623,-22.));
#115240=CARTESIAN_POINT('',(-9.06658668237251,24.4862266006622,-22.));
#115241=CARTESIAN_POINT('',(-9.06658668237251,24.4862266006622,-22.));
#115242=CARTESIAN_POINT('Origin',(-9.06658668237251,24.2952266006623,-22.));
#115243=CARTESIAN_POINT('',(-21.234,0.12950000000008,-22.));
#115244=CARTESIAN_POINT('Origin',(-18.734,0.12950000000008,-22.));
#115245=CARTESIAN_POINT('',(16.234,0.12950000000008,-22.));
#115246=CARTESIAN_POINT('Origin',(18.734,0.12950000000008,-22.));
#115247=CARTESIAN_POINT('Ctrl Pts',(-17.1140743056112,17.8480877707428,
-22.));
#115248=CARTESIAN_POINT('Ctrl Pts',(-17.0603911270984,17.8998883320905,
-22.));
#115249=CARTESIAN_POINT('Ctrl Pts',(-17.0098645090452,17.954561484389,-22.));
#115250=CARTESIAN_POINT('Ctrl Pts',(-16.9624881824911,18.0117359214698,
-22.));
#115251=CARTESIAN_POINT('Ctrl Pts',(-16.9134245435091,18.0709466316275,
-22.));
#115252=CARTESIAN_POINT('Ctrl Pts',(-16.8677390829668,18.1328404012573,
-22.));
#115253=CARTESIAN_POINT('Ctrl Pts',(-16.8254531772989,18.1970544303157,
-22.));
#115254=CARTESIAN_POINT('Ctrl Pts',(-16.7853186877899,18.2580013873422,
-22.));
#115255=CARTESIAN_POINT('Ctrl Pts',(-16.7482465752162,18.3210394463055,
-22.));
#115256=CARTESIAN_POINT('Ctrl Pts',(-16.7142835835435,18.3858911656733,
-22.));
#115257=CARTESIAN_POINT('Ctrl Pts',(-16.6991852702862,18.414721122225,-22.));
#115258=CARTESIAN_POINT('Ctrl Pts',(-16.6847017945038,18.443909871674,-22.));
#115259=CARTESIAN_POINT('Ctrl Pts',(-16.6708392558117,18.4734345779294,
-22.));
#115260=CARTESIAN_POINT('Ctrl Pts',(-16.6640109132328,18.4879777156138,
-22.));
#115261=CARTESIAN_POINT('Ctrl Pts',(-16.6573332485221,18.5026023792008,
-22.));
#115262=CARTESIAN_POINT('Ctrl Pts',(-16.6508071085471,18.5173059065043,
-22.));
#115263=CARTESIAN_POINT('Ctrl Pts',(-16.6447949281281,18.53085147238,-22.));
#115264=CARTESIAN_POINT('Ctrl Pts',(-16.638910878667,18.5444653615358,-22.));
#115265=CARTESIAN_POINT('Ctrl Pts',(-16.6331635636444,18.5581259521741,
-22.));
#115266=CARTESIAN_POINT('Ctrl Pts',(-16.6020947551997,18.6319723086221,
-22.));
#115267=CARTESIAN_POINT('Ctrl Pts',(-16.5749611536668,18.7073070289839,
-22.));
#115268=CARTESIAN_POINT('Ctrl Pts',(-16.5517843887068,18.7837489743025,
-22.));
#115269=CARTESIAN_POINT('Ctrl Pts',(-16.5281812491805,18.8615971944543,
-22.));
#115270=CARTESIAN_POINT('Ctrl Pts',(-16.5086813563681,18.9405945618165,
-22.));
#115271=CARTESIAN_POINT('Ctrl Pts',(-16.4933484509613,19.0203740751675,
-22.));
#115272=CARTESIAN_POINT('Ctrl Pts',(-16.4794162132308,19.0928656947625,
-22.));
#115273=CARTESIAN_POINT('Ctrl Pts',(-16.4689246908346,19.1660040425392,
-22.));
#115274=CARTESIAN_POINT('Ctrl Pts',(-16.461955492605,19.2395296145576,-22.));
#115275=CARTESIAN_POINT('Ctrl Pts',(-16.4592975702873,19.2675708974063,
-22.));
#115276=CARTESIAN_POINT('Ctrl Pts',(-16.4571523310073,19.2956686091404,
-22.));
#115277=CARTESIAN_POINT('Ctrl Pts',(-16.4555256621827,19.3238086400899,
-22.));
#115278=CARTESIAN_POINT('Ctrl Pts',(-16.4546321787531,19.3392651675542,
-22.));
#115279=CARTESIAN_POINT('Ctrl Pts',(-16.4538951614737,19.3547344644167,
-22.));
#115280=CARTESIAN_POINT('Ctrl Pts',(-16.4533156881431,19.3702141998337,
-22.));
#115281=CARTESIAN_POINT('Ctrl Pts',(-16.4528679850542,19.3821738966753,
-22.));
#115282=CARTESIAN_POINT('Ctrl Pts',(-16.4525144924858,19.3941365263619,
-22.));
#115283=CARTESIAN_POINT('Ctrl Pts',(-16.452255631388,19.4060924704157,-22.));
#115284=CARTESIAN_POINT('Ctrl Pts',(-16.4504487968614,19.4895442238956,
-22.));
#115285=CARTESIAN_POINT('Ctrl Pts',(-16.4532437926239,19.5727897376045,
-22.));
#115286=CARTESIAN_POINT('Ctrl Pts',(-16.4606968610006,19.6554483758564,
-22.));
#115287=CARTESIAN_POINT('Ctrl Pts',(-16.4681356985408,19.7379491862844,
-22.));
#115288=CARTESIAN_POINT('Ctrl Pts',(-16.4802144629511,19.8198663642554,
-22.));
#115289=CARTESIAN_POINT('Ctrl Pts',(-16.4970384375915,19.9008370756969,
-22.));
#115290=CARTESIAN_POINT('Ctrl Pts',(-16.5135067566735,19.9800960820143,
-22.));
#115291=CARTESIAN_POINT('Ctrl Pts',(-16.5345215459181,20.058449172967,-22.));
#115292=CARTESIAN_POINT('Ctrl Pts',(-16.5598157066501,20.135668594405,-22.));
#115293=CARTESIAN_POINT('Ctrl Pts',(-16.5701726792029,20.1672869365532,
-22.));
#115294=CARTESIAN_POINT('Ctrl Pts',(-16.5812477391057,20.1987151389824,
-22.));
#115295=CARTESIAN_POINT('Ctrl Pts',(-16.5930250010084,20.2299370972628,
-22.));
#115296=CARTESIAN_POINT('Ctrl Pts',(-16.5995762661519,20.2473047442324,
-22.));
#115297=CARTESIAN_POINT('Ctrl Pts',(-16.6063470587533,20.2646137128558,
-22.));
#115298=CARTESIAN_POINT('Ctrl Pts',(-16.6133222512795,20.2818311531004,
-22.));
#115299=CARTESIAN_POINT('Ctrl Pts',(-16.644281419466,20.3582502091005,-22.));
#115300=CARTESIAN_POINT('Ctrl Pts',(-16.6792964912941,20.432962513728,-22.));
#115301=CARTESIAN_POINT('Ctrl Pts',(-16.7180394494849,20.5057444546798,
-22.));
#115302=CARTESIAN_POINT('Ctrl Pts',(-16.7588463546246,20.5824036954551,
-22.));
#115303=CARTESIAN_POINT('Ctrl Pts',(-16.8037889572456,20.6569222708542,
-22.));
#115304=CARTESIAN_POINT('Ctrl Pts',(-16.8525444691545,20.7290332608009,
-22.));
#115305=CARTESIAN_POINT('Ctrl Pts',(-16.9012999810635,20.8011442507477,
-22.));
#115306=CARTESIAN_POINT('Ctrl Pts',(-16.9538690009003,20.8708485410036,
-22.));
#115307=CARTESIAN_POINT('Ctrl Pts',(-17.0099819921104,20.9378605149736,
-22.));
#115308=CARTESIAN_POINT('Ctrl Pts',(-17.0318957015214,20.9640305852723,
-22.));
#115309=CARTESIAN_POINT('Ctrl Pts',(-17.0543504354563,20.9897897710343,
-22.));
#115310=CARTESIAN_POINT('Ctrl Pts',(-17.0773320398146,21.0151198306804,
-22.));
#115311=CARTESIAN_POINT('Ctrl Pts',(-17.08646379095,21.0251847416122,-22.));
#115312=CARTESIAN_POINT('Ctrl Pts',(-17.0956794941242,21.0351826951285,
-22.));
#115313=CARTESIAN_POINT('Ctrl Pts',(-17.1049759541041,21.045110003522,-22.));
#115314=CARTESIAN_POINT('Ctrl Pts',(-17.1654855277221,21.1097256958788,
-22.));
#115315=CARTESIAN_POINT('Ctrl Pts',(-17.2292148909452,21.171140300117,-22.));
#115316=CARTESIAN_POINT('Ctrl Pts',(-17.2958559579295,21.2290794537635,
-22.));
#115317=CARTESIAN_POINT('Ctrl Pts',(-17.3510488196551,21.2770652955339,
-22.));
#115318=CARTESIAN_POINT('Ctrl Pts',(-17.4082400388151,21.3226671775257,
-22.));
#115319=CARTESIAN_POINT('Ctrl Pts',(-17.4672777521355,21.3657152682276,
-22.));
#115320=CARTESIAN_POINT('Ctrl Pts',(-17.4867746843808,21.3799317014277,
-22.));
#115321=CARTESIAN_POINT('Ctrl Pts',(-17.5064731515178,21.3938694861353,
-22.));
#115322=CARTESIAN_POINT('Ctrl Pts',(-17.5263681121617,21.4075220975473,
-22.));
#115323=CARTESIAN_POINT('Ctrl Pts',(-17.542293137778,21.4184504019736,-22.));
#115324=CARTESIAN_POINT('Ctrl Pts',(-17.55834542777,21.429196741247,-22.));
#115325=CARTESIAN_POINT('Ctrl Pts',(-17.5745064519429,21.439747587913,-22.));
#115326=CARTESIAN_POINT('Ctrl Pts',(-17.6490342197562,21.4884036039023,
-22.));
#115327=CARTESIAN_POINT('Ctrl Pts',(-17.7259441256673,21.5329559340006,
-22.));
#115328=CARTESIAN_POINT('Ctrl Pts',(-17.8049553049308,21.5731139747841,
-22.));
#115329=CARTESIAN_POINT('Ctrl Pts',(-17.8827965257828,21.6126773751883,
-22.));
#115330=CARTESIAN_POINT('Ctrl Pts',(-17.9626779315913,21.6479763829434,
-22.));
#115331=CARTESIAN_POINT('Ctrl Pts',(-18.0443633906767,21.6786957524571,
-22.));
#115332=CARTESIAN_POINT('Ctrl Pts',(-18.0530581575347,21.6819655847986,
-22.));
#115333=CARTESIAN_POINT('Ctrl Pts',(-18.0617733892786,21.6851834888842,
-22.));
#115334=CARTESIAN_POINT('Ctrl Pts',(-18.070508670429,21.6883495949495,-22.));
#115335=CARTESIAN_POINT('Ctrl Pts',(-19.3957372685686,21.6839949024184,
-22.));
#115336=CARTESIAN_POINT('Ctrl Pts',(-19.477389057327,21.6544306829991,-22.));
#115337=CARTESIAN_POINT('Ctrl Pts',(-19.5571491338507,21.6204660242302,
-22.));
#115338=CARTESIAN_POINT('Ctrl Pts',(-19.6348154715244,21.5824187572536,
-22.));
#115339=CARTESIAN_POINT('Ctrl Pts',(-19.7143271161377,21.5434675093776,
-22.));
#115340=CARTESIAN_POINT('Ctrl Pts',(-19.7916450682551,21.5002366973253,
-22.));
#115341=CARTESIAN_POINT('Ctrl Pts',(-19.8665231148743,21.4530209100808,
-22.));
#115342=CARTESIAN_POINT('Ctrl Pts',(-19.9365885412315,21.4088398127707,
-22.));
#115343=CARTESIAN_POINT('Ctrl Pts',(-20.0045177600144,21.3611685582697,
-22.));
#115344=CARTESIAN_POINT('Ctrl Pts',(-20.0700782126376,21.3102210028104,
-22.));
#115345=CARTESIAN_POINT('Ctrl Pts',(-20.0997466183463,21.2871654459197,
-22.));
#115346=CARTESIAN_POINT('Ctrl Pts',(-20.1289294820831,21.2634386377592,
-22.));
#115347=CARTESIAN_POINT('Ctrl Pts',(-20.1576028623549,21.2390591151444,
-22.));
#115348=CARTESIAN_POINT('Ctrl Pts',(-20.1753080822265,21.2240052636568,
-22.));
#115349=CARTESIAN_POINT('Ctrl Pts',(-20.1928190152044,21.2087025308569,
-22.));
#115350=CARTESIAN_POINT('Ctrl Pts',(-20.2101297112266,21.1931551680194,
-22.));
#115351=CARTESIAN_POINT('Ctrl Pts',(-20.222291744835,21.182232005305,-22.));
#115352=CARTESIAN_POINT('Ctrl Pts',(-20.2343567146449,21.1711862914419,
-22.));
#115353=CARTESIAN_POINT('Ctrl Pts',(-20.2463056588354,21.1600355900683,
-22.));
#115354=CARTESIAN_POINT('Ctrl Pts',(-20.3097374358009,21.1008413389894,
-22.));
#115355=CARTESIAN_POINT('Ctrl Pts',(-20.3700068738243,21.0385997406358,
-22.));
#115356=CARTESIAN_POINT('Ctrl Pts',(-20.4268834135291,20.9735889911136,
-22.));
#115357=CARTESIAN_POINT('Ctrl Pts',(-20.4830375566033,20.9094039519221,
-22.));
#115358=CARTESIAN_POINT('Ctrl Pts',(-20.5358848927175,20.8425188203043,
-22.));
#115359=CARTESIAN_POINT('Ctrl Pts',(-20.5851610183652,20.7731751875981,
-22.));
#115360=CARTESIAN_POINT('Ctrl Pts',(-20.6305982452152,20.7092338300246,
-22.));
#115361=CARTESIAN_POINT('Ctrl Pts',(-20.6729988898206,20.6432013951078,
-22.));
#115362=CARTESIAN_POINT('Ctrl Pts',(-20.7121179614365,20.5752560755747,
-22.0000000000001));
#115363=CARTESIAN_POINT('Ctrl Pts',(-20.7284900120376,20.5468197103046,
-22.0000000000001));
#115364=CARTESIAN_POINT('Ctrl Pts',(-20.7442868026563,20.5180482040854,
-22.));
#115365=CARTESIAN_POINT('Ctrl Pts',(-20.7594882606863,20.4889543859677,
-22.));
#115366=CARTESIAN_POINT('Ctrl Pts',(-20.769344952432,20.4700898272965,-22.));
#115367=CARTESIAN_POINT('Ctrl Pts',(-20.7789513234994,20.4510897578356,
-22.));
#115368=CARTESIAN_POINT('Ctrl Pts',(-20.7883016018661,20.4319576715327,
-22.));
#115369=CARTESIAN_POINT('Ctrl Pts',(-20.7942275528717,20.4198322778685,
-22.));
#115370=CARTESIAN_POINT('Ctrl Pts',(-20.800046810587,20.4076616313445,-22.));
#115371=CARTESIAN_POINT('Ctrl Pts',(-20.8057567064001,20.3954502940177,
-22.));
#115372=CARTESIAN_POINT('Ctrl Pts',(-20.8408822399145,20.3203298798152,
-22.));
#115373=CARTESIAN_POINT('Ctrl Pts',(-20.8718943362061,20.2436277257691,
-22.));
#115374=CARTESIAN_POINT('Ctrl Pts',(-20.898546197771,20.1655724028405,-22.));
#115375=CARTESIAN_POINT('Ctrl Pts',(-20.9251980593358,20.0875170799122,
-22.));
#115376=CARTESIAN_POINT('Ctrl Pts',(-20.9474901582818,20.008107858314,-22.));
#115377=CARTESIAN_POINT('Ctrl Pts',(-20.9651213884777,19.9275640466204,
-22.));
#115378=CARTESIAN_POINT('Ctrl Pts',(-20.982945860616,19.8461374580334,-22.));
#115379=CARTESIAN_POINT('Ctrl Pts',(-20.9960059981342,19.7635500467728,
-22.));
#115380=CARTESIAN_POINT('Ctrl Pts',(-21.0043774598022,19.6801932612386,
-22.));
#115381=CARTESIAN_POINT('Ctrl Pts',(-21.0078359299807,19.6457563888755,
-22.));
#115382=CARTESIAN_POINT('Ctrl Pts',(-21.0104935728588,19.6111883610475,
-22.));
#115383=CARTESIAN_POINT('Ctrl Pts',(-21.0123533015418,19.5765177064329,
-22.));
#115384=CARTESIAN_POINT('Ctrl Pts',(-21.01308526083,19.5628718945969,-22.));
#115385=CARTESIAN_POINT('Ctrl Pts',(-21.0136936024307,19.5492081941022,
-22.));
#115386=CARTESIAN_POINT('Ctrl Pts',(-21.0141780332164,19.535546001816,-22.));
#115387=CARTESIAN_POINT('Ctrl Pts',(-21.0170628012175,19.4541881354373,
-22.));
#115388=CARTESIAN_POINT('Ctrl Pts',(-21.0155662532645,19.372753622897,-22.));
#115389=CARTESIAN_POINT('Ctrl Pts',(-21.009821014486,19.2915996489843,-22.));
#115390=CARTESIAN_POINT('Ctrl Pts',(-21.0040551150003,19.2101538336792,
-22.));
#115391=CARTESIAN_POINT('Ctrl Pts',(-20.9940095377782,19.1289895606253,
-22.));
#115392=CARTESIAN_POINT('Ctrl Pts',(-20.9797676620298,19.0484794559438,
-22.));
#115393=CARTESIAN_POINT('Ctrl Pts',(-20.9656474978692,18.9686573935437,
-22.));
#115394=CARTESIAN_POINT('Ctrl Pts',(-20.9474020142807,18.8894774430529,
-22.));
#115395=CARTESIAN_POINT('Ctrl Pts',(-20.9250689442011,18.8113285395616,
-22.));
#115396=CARTESIAN_POINT('Ctrl Pts',(-20.915771730189,18.7787953017227,-22.));
#115397=CARTESIAN_POINT('Ctrl Pts',(-20.9057656352848,18.7464411369984,
-22.));
#115398=CARTESIAN_POINT('Ctrl Pts',(-20.8950513997073,18.714296014732,-22.));
#115399=CARTESIAN_POINT('Ctrl Pts',(-20.8895107302012,18.6976727570651,
-22.));
#115400=CARTESIAN_POINT('Ctrl Pts',(-20.8837798036466,18.681103370745,-22.));
#115401=CARTESIAN_POINT('Ctrl Pts',(-20.8778666056241,18.6646133670345,
-22.));
#115402=CARTESIAN_POINT('Ctrl Pts',(-20.8511334433403,18.5900631923957,
-22.));
#115403=CARTESIAN_POINT('Ctrl Pts',(-20.8206474037361,18.5170371727757,
-22.));
#115404=CARTESIAN_POINT('Ctrl Pts',(-20.7864673395051,18.4458945668894,
-22.));
#115405=CARTESIAN_POINT('Ctrl Pts',(-20.7601551393027,18.3911281838789,
-22.));
#115406=CARTESIAN_POINT('Ctrl Pts',(-20.7316529155262,18.3374783045939,
-21.9999999999999));
#115407=CARTESIAN_POINT('Ctrl Pts',(-20.7009723139099,18.2851235072403,
-22.));
#115408=CARTESIAN_POINT('Ctrl Pts',(-20.6917380438118,18.2693657217269,
-22.));
#115409=CARTESIAN_POINT('Ctrl Pts',(-20.6823063515041,18.2537253600017,
-22.));
#115410=CARTESIAN_POINT('Ctrl Pts',(-20.6726773431573,18.2382075723836,
-21.9999999999999));
#115411=CARTESIAN_POINT('Ctrl Pts',(-20.6644524248536,18.2249525692911,
-21.9999999999999));
#115412=CARTESIAN_POINT('Ctrl Pts',(-20.6560858067932,18.2117907655657,
-22.));
#115413=CARTESIAN_POINT('Ctrl Pts',(-20.6475820990968,18.1987316736659,
-22.));
#115414=CARTESIAN_POINT('Ctrl Pts',(-20.6064305731469,18.1355355269518,
-22.));
#115415=CARTESIAN_POINT('Ctrl Pts',(-20.562041925838,18.0746943297042,-22.));
#115416=CARTESIAN_POINT('Ctrl Pts',(-20.5144495325811,18.0165478115783,
-22.));
#115417=CARTESIAN_POINT('Ctrl Pts',(-20.4703173158396,17.9626288013103,
-21.9999999999999));
#115418=CARTESIAN_POINT('Ctrl Pts',(-20.4234297243619,17.9110267653547,
-22.));
#115419=CARTESIAN_POINT('Ctrl Pts',(-20.3737908005412,17.8620457668345,
-22.));
#115420=CARTESIAN_POINT('Ctrl Pts',(-20.368202240041,17.8565312783541,-22.));
#115421=CARTESIAN_POINT('Ctrl Pts',(-20.3625787852046,17.8510500502091,
-22.));
#115422=CARTESIAN_POINT('Ctrl Pts',(-20.3569208045551,17.8456022314362,
-21.9999999999999));
#115423=CARTESIAN_POINT('Ctrl Pts',(20.3539256943888,17.8480877707428,-22.));
#115424=CARTESIAN_POINT('Ctrl Pts',(20.4076088569716,17.8998883167192,-22.));
#115425=CARTESIAN_POINT('Ctrl Pts',(20.458135458206,17.9545614547721,-22.));
#115426=CARTESIAN_POINT('Ctrl Pts',(20.5055117676562,18.0117358784471,-22.));
#115427=CARTESIAN_POINT('Ctrl Pts',(20.5545753925304,18.0709465790724,-22.));
#115428=CARTESIAN_POINT('Ctrl Pts',(20.6002608381613,18.1328403404639,-22.));
#115429=CARTESIAN_POINT('Ctrl Pts',(20.6425467287669,18.1970543621741,-22.));
#115430=CARTESIAN_POINT('Ctrl Pts',(20.6826812143677,18.2580013280008,-22.));
#115431=CARTESIAN_POINT('Ctrl Pts',(20.719753321312,18.3210393976475,-22.));
#115432=CARTESIAN_POINT('Ctrl Pts',(20.7537163061537,18.3858911290265,-22.));
#115433=CARTESIAN_POINT('Ctrl Pts',(20.7688146169019,18.4147210919254,-22.));
#115434=CARTESIAN_POINT('Ctrl Pts',(20.7832980898944,18.4439098480094,-22.));
#115435=CARTESIAN_POINT('Ctrl Pts',(20.79716062556,18.4734345611379,-22.));
#115436=CARTESIAN_POINT('Ctrl Pts',(20.8039889483082,18.4879776631471,-22.));
#115437=CARTESIAN_POINT('Ctrl Pts',(20.8106665939401,18.5026022906791,-22.));
#115438=CARTESIAN_POINT('Ctrl Pts',(20.8171927156004,18.5173057815627,-22.));
#115439=CARTESIAN_POINT('Ctrl Pts',(20.8232049158819,18.5308513966511,-22.));
#115440=CARTESIAN_POINT('Ctrl Pts',(20.8290889843231,18.5444653356248,-22.));
#115441=CARTESIAN_POINT('Ctrl Pts',(20.834836317356,18.5581259764514,-22.));
#115442=CARTESIAN_POINT('Ctrl Pts',(20.8659051086395,18.6319723320064,-22.));
#115443=CARTESIAN_POINT('Ctrl Pts',(20.8930386939032,18.7073070517052,-22.));
#115444=CARTESIAN_POINT('Ctrl Pts',(20.9162154441631,18.7837489961395,-22.));
#115445=CARTESIAN_POINT('Ctrl Pts',(20.9398185727455,18.8615972286714,-22.));
#115446=CARTESIAN_POINT('Ctrl Pts',(20.9593184548407,18.9405946085753,-22.));
#115447=CARTESIAN_POINT('Ctrl Pts',(20.9746513504475,19.0203741339709,-22.));
#115448=CARTESIAN_POINT('Ctrl Pts',(20.9885835808443,19.0928657726845,-22.));
#115449=CARTESIAN_POINT('Ctrl Pts',(20.9990750958876,19.1660041393162,-22.));
#115450=CARTESIAN_POINT('Ctrl Pts',(21.0060442872368,19.2395297293499,-22.));
#115451=CARTESIAN_POINT('Ctrl Pts',(21.0087022058165,19.2675710073175,-22.));
#115452=CARTESIAN_POINT('Ctrl Pts',(21.0108474418568,19.2956687140012,-22.));
#115453=CARTESIAN_POINT('Ctrl Pts',(21.0124741079748,19.3238087397167,-22.));
#115454=CARTESIAN_POINT('Ctrl Pts',(21.0133675811686,19.3392651129519,-22.));
#115455=CARTESIAN_POINT('Ctrl Pts',(21.0141045914371,19.3547342552799,-22.));
#115456=CARTESIAN_POINT('Ctrl Pts',(21.0146840610199,19.370213835923,-22.));
#115457=CARTESIAN_POINT('Ctrl Pts',(21.0151317606382,19.3821733978234,-22.));
#115458=CARTESIAN_POINT('Ctrl Pts',(21.0154852519447,19.3941358929903,-22.));
#115459=CARTESIAN_POINT('Ctrl Pts',(21.0157441139737,19.4060917025175,-22.));
#115460=CARTESIAN_POINT('Ctrl Pts',(21.0175509756949,19.4895434728017,-22.));
#115461=CARTESIAN_POINT('Ctrl Pts',(21.0147560087132,19.5727890030198,-22.));
#115462=CARTESIAN_POINT('Ctrl Pts',(21.0073029715582,19.655447656657,-22.));
#115463=CARTESIAN_POINT('Ctrl Pts',(20.9998641358153,19.737948808113,-22.));
#115464=CARTESIAN_POINT('Ctrl Pts',(20.987785339035,19.819866321382,-22.));
#115465=CARTESIAN_POINT('Ctrl Pts',(20.9709612973755,19.9008373573407,-22.));
#115466=CARTESIAN_POINT('Ctrl Pts',(20.9545235681866,19.9799491420218,-22.));
#115467=CARTESIAN_POINT('Ctrl Pts',(20.933556230191,20.0581583683546,-22.));
#115468=CARTESIAN_POINT('Ctrl Pts',(20.9083249440286,20.1352385562694,-22.));
#115469=CARTESIAN_POINT('Ctrl Pts',(20.8979275365846,20.1670020626737,-22.));
#115470=CARTESIAN_POINT('Ctrl Pts',(20.886805437583,20.198573773065,-22.));
#115471=CARTESIAN_POINT('Ctrl Pts',(20.8749747526326,20.2299373637517,-22.));
#115472=CARTESIAN_POINT('Ctrl Pts',(20.8684234889834,20.2473050100404,-22.));
#115473=CARTESIAN_POINT('Ctrl Pts',(20.8616526979763,20.2646139778576,-22.));
#115474=CARTESIAN_POINT('Ctrl Pts',(20.854677507136,20.2818314171768,-22.));
#115475=CARTESIAN_POINT('Ctrl Pts',(20.8237183426601,20.3582504783803,-22.));
#115476=CARTESIAN_POINT('Ctrl Pts',(20.7887032753635,20.4329627854485,-22.));
#115477=CARTESIAN_POINT('Ctrl Pts',(20.7499603220885,20.5057447265529,-22.));
#115478=CARTESIAN_POINT('Ctrl Pts',(20.7091534306779,20.5824039514244,-22.));
#115479=CARTESIAN_POINT('Ctrl Pts',(20.6642108439443,20.6569225092783,-22.));
#115480=CARTESIAN_POINT('Ctrl Pts',(20.6154553493761,20.7290334807154,-22.));
#115481=CARTESIAN_POINT('Ctrl Pts',(20.5666998548079,20.8011444521525,-22.));
#115482=CARTESIAN_POINT('Ctrl Pts',(20.5141308537666,20.8708487229331,-22.));
#115483=CARTESIAN_POINT('Ctrl Pts',(20.4580178821339,20.9378606771181,-22.));
#115484=CARTESIAN_POINT('Ctrl Pts',(20.4361041795504,20.9640307406671,-22.));
#115485=CARTESIAN_POINT('Ctrl Pts',(20.4136494525221,20.9897899196015,-22.));
#115486=CARTESIAN_POINT('Ctrl Pts',(20.3906678551117,21.0151199723788,-22.));
#115487=CARTESIAN_POINT('Ctrl Pts',(20.3815361086865,21.0251848784325,-22.));
#115488=CARTESIAN_POINT('Ctrl Pts',(20.3723204102617,21.0351828270963,-22.));
#115489=CARTESIAN_POINT('Ctrl Pts',(20.3630239550768,21.0451101306559,-22.));
#115490=CARTESIAN_POINT('Ctrl Pts',(20.3025143985113,21.1097258066671,-22.));
#115491=CARTESIAN_POINT('Ctrl Pts',(20.2387850522984,21.1711403943427,-22.));
#115492=CARTESIAN_POINT('Ctrl Pts',(20.1721440016479,21.2290795318307,-22.));
#115493=CARTESIAN_POINT('Ctrl Pts',(20.1169511545801,21.277065359236,-22.));
#115494=CARTESIAN_POINT('Ctrl Pts',(20.0597599496963,21.3226672272365,-22.));
#115495=CARTESIAN_POINT('Ctrl Pts',(20.0007222499054,21.3657153046774,-22.));
#115496=CARTESIAN_POINT('Ctrl Pts',(19.9812253064434,21.3799317449347,-22.));
#115497=CARTESIAN_POINT('Ctrl Pts',(19.9615268276842,21.3938695363309,-22.));
#115498=CARTESIAN_POINT('Ctrl Pts',(19.9416318550109,21.4075221540601,-22.));
#115499=CARTESIAN_POINT('Ctrl Pts',(19.9257068576964,21.4184504375137,-22.));
#115500=CARTESIAN_POINT('Ctrl Pts',(19.9096545963614,21.4291967564363,-22.));
#115501=CARTESIAN_POINT('Ctrl Pts',(19.8934936011196,21.4397475834371,-22.));
#115502=CARTESIAN_POINT('Ctrl Pts',(19.8189658486552,21.4884035858209,-22.));
#115503=CARTESIAN_POINT('Ctrl Pts',(19.7420559565434,21.5329559037425,-22.));
#115504=CARTESIAN_POINT('Ctrl Pts',(19.6630447888977,21.5731139344032,-22.));
#115505=CARTESIAN_POINT('Ctrl Pts',(19.5852035756509,21.6126773267864,-22.));
#115506=CARTESIAN_POINT('Ctrl Pts',(19.5053221751299,21.6479763280926,-22.));
#115507=CARTESIAN_POINT('Ctrl Pts',(19.423636718432,21.6786956932901,-22.));
#115508=CARTESIAN_POINT('Ctrl Pts',(19.414941951073,21.6819655254562,-22.));
#115509=CARTESIAN_POINT('Ctrl Pts',(19.4062267187917,21.6851834293815,-22.));
#115510=CARTESIAN_POINT('Ctrl Pts',(19.3974914370682,21.6883495353011,-22.));
#115511=CARTESIAN_POINT('Ctrl Pts',(18.0722627314313,21.6839949024184,-22.));
#115512=CARTESIAN_POINT('Ctrl Pts',(17.9906108868453,21.6544306627852,-22.));
#115513=CARTESIAN_POINT('Ctrl Pts',(17.9108507545872,21.6204659928942,-22.));
#115514=CARTESIAN_POINT('Ctrl Pts',(17.8331843622587,21.5824187212757,-22.));
#115515=CARTESIAN_POINT('Ctrl Pts',(17.7536727057571,21.5434674902341,-22.));
#115516=CARTESIAN_POINT('Ctrl Pts',(17.6763547404512,21.5002367065515,-22.));
#115517=CARTESIAN_POINT('Ctrl Pts',(17.6014766800473,21.4530209559463,-22.));
#115518=CARTESIAN_POINT('Ctrl Pts',(17.53141126818,21.408839910191,-22.));
#115519=CARTESIAN_POINT('Ctrl Pts',(17.4634820616961,21.361168717218,-22.));
#115520=CARTESIAN_POINT('Ctrl Pts',(17.3979216194972,21.3102212303572,-22.));
#115521=CARTESIAN_POINT('Ctrl Pts',(17.3682532365539,21.287165718535,-22.));
#115522=CARTESIAN_POINT('Ctrl Pts',(17.3390703946074,21.2634389577077,-22.));
#115523=CARTESIAN_POINT('Ctrl Pts',(17.3103970351346,21.2390594843875,-22.));
#115524=CARTESIAN_POINT('Ctrl Pts',(17.2926918259638,21.2240056615169,-22.));
#115525=CARTESIAN_POINT('Ctrl Pts',(17.2751809033557,21.2087029580218,-22.));
#115526=CARTESIAN_POINT('Ctrl Pts',(17.2578702173692,21.1931556251064,-22.));
#115527=CARTESIAN_POINT('Ctrl Pts',(17.2457081795529,21.1822324733025,-22.));
#115528=CARTESIAN_POINT('Ctrl Pts',(17.2336432055526,21.1711867704329,-22.));
#115529=CARTESIAN_POINT('Ctrl Pts',(17.2216942572027,21.160036080102,-22.));
#115530=CARTESIAN_POINT('Ctrl Pts',(17.1582624698647,21.1008418985699,-22.));
#115531=CARTESIAN_POINT('Ctrl Pts',(17.0979930211183,21.0386003723497,-22.));
#115532=CARTESIAN_POINT('Ctrl Pts',(17.0411164708952,20.973589694329,-22.));
#115533=CARTESIAN_POINT('Ctrl Pts',(16.9849623314079,20.9094047417006,-22.));
#115534=CARTESIAN_POINT('Ctrl Pts',(16.9321149974354,20.842519697379,-22.));
#115535=CARTESIAN_POINT('Ctrl Pts',(16.8828388728193,20.7731761494008,-22.));
#115536=CARTESIAN_POINT('Ctrl Pts',(16.8374016308099,20.7092348472829,-22.));
#115537=CARTESIAN_POINT('Ctrl Pts',(16.7950009722518,20.6432024641596,-22.));
#115538=CARTESIAN_POINT('Ctrl Pts',(16.7558818883965,20.5752571902803,-22.));
#115539=CARTESIAN_POINT('Ctrl Pts',(16.7395098281522,20.5468208362648,-22.));
#115540=CARTESIAN_POINT('Ctrl Pts',(16.7237130285085,20.5180493400384,-22.));
#115541=CARTESIAN_POINT('Ctrl Pts',(16.7085115621276,20.4889555304732,-22.));
#115542=CARTESIAN_POINT('Ctrl Pts',(16.6986548604459,20.4700909686944,-22.));
#115543=CARTESIAN_POINT('Ctrl Pts',(16.6890484799558,20.4510908953963,-22.));
#115544=CARTESIAN_POINT('Ctrl Pts',(16.6796981927033,20.4319588044811,-22.));
#115545=CARTESIAN_POINT('Ctrl Pts',(16.6737722459446,20.4198334281067,-22.));
#115546=CARTESIAN_POINT('Ctrl Pts',(16.6679529923645,20.4076627987652,-22.));
#115547=CARTESIAN_POINT('Ctrl Pts',(16.6622431005404,20.3954514784257,-22.));
#115548=CARTESIAN_POINT('Ctrl Pts',(16.6271175635218,20.3203311087503,-22.));
#115549=CARTESIAN_POINT('Ctrl Pts',(16.5961054651676,20.2436289901797,-22.));
#115550=CARTESIAN_POINT('Ctrl Pts',(16.5694536034806,20.1655736906577,-22.));
#115551=CARTESIAN_POINT('Ctrl Pts',(16.5428017417936,20.087518391136,-22.));
#115552=CARTESIAN_POINT('Ctrl Pts',(16.5205096446651,20.0081091808815,-22.));
#115553=CARTESIAN_POINT('Ctrl Pts',(16.5028784187468,19.9275653652902,-22.));
#115554=CARTESIAN_POINT('Ctrl Pts',(16.4850539498385,19.8461387677624,-22.));
#115555=CARTESIAN_POINT('Ctrl Pts',(16.4719938186516,19.7635513318282,-22.));
#115556=CARTESIAN_POINT('Ctrl Pts',(16.4636223658545,19.6801945089039,-22.));
#115557=CARTESIAN_POINT('Ctrl Pts',(16.4601638998612,19.6457576262764,-22.));
#115558=CARTESIAN_POINT('Ctrl Pts',(16.457506261361,19.6111895860526,-22.));
#115559=CARTESIAN_POINT('Ctrl Pts',(16.4556465372103,19.5765189171097,-22.));
#115560=CARTESIAN_POINT('Ctrl Pts',(16.4549145796191,19.5628730980147,-22.));
#115561=CARTESIAN_POINT('Ctrl Pts',(16.4543062397689,19.5492093899537,-22.));
#115562=CARTESIAN_POINT('Ctrl Pts',(16.4538218107824,19.535547189819,-22.));
#115563=CARTESIAN_POINT('Ctrl Pts',(16.450937053514,19.4541892772202,-22.));
#115564=CARTESIAN_POINT('Ctrl Pts',(16.4524336138896,19.3727547084354,-22.));
#115565=CARTESIAN_POINT('Ctrl Pts',(16.4581788662374,19.291600671179,-22.));
#115566=CARTESIAN_POINT('Ctrl Pts',(16.4639447791335,19.210154795236,-22.));
#115567=CARTESIAN_POINT('Ctrl Pts',(16.4739903706141,19.128990454367,-22.));
#115568=CARTESIAN_POINT('Ctrl Pts',(16.4882322609366,19.0484802775444,-22.));
#115569=CARTESIAN_POINT('Ctrl Pts',(16.502352437732,18.9686581538777,-22.));
#115570=CARTESIAN_POINT('Ctrl Pts',(16.520597933207,18.8894781376979,-22.));
#115571=CARTESIAN_POINT('Ctrl Pts',(16.5429310139029,18.8113291667476,-22.));
#115572=CARTESIAN_POINT('Ctrl Pts',(16.5522282344977,18.7787958932563,-22.));
#115573=CARTESIAN_POINT('Ctrl Pts',(16.5622343360937,18.7464416926568,-21.9999999999999));
#115574=CARTESIAN_POINT('Ctrl Pts',(16.5729485784318,18.7142965345087,-22.));
#115575=CARTESIAN_POINT('Ctrl Pts',(16.5784892537261,18.6976732514091,-22.));
#115576=CARTESIAN_POINT('Ctrl Pts',(16.5842201862524,18.6811038396758,-22.));
#115577=CARTESIAN_POINT('Ctrl Pts',(16.5901333904085,18.6646138106646,-22.));
#115578=CARTESIAN_POINT('Ctrl Pts',(16.6168665610553,18.5900635756494,-22.));
#115579=CARTESIAN_POINT('Ctrl Pts',(16.6473526068873,18.5170374956828,-22.));
#115580=CARTESIAN_POINT('Ctrl Pts',(16.6815326747322,18.4458948319453,-22.));
#115581=CARTESIAN_POINT('Ctrl Pts',(16.7078448953081,18.3911283677852,-22.));
#115582=CARTESIAN_POINT('Ctrl Pts',(16.7363471408355,18.3374784103201,-22.));
#115583=CARTESIAN_POINT('Ctrl Pts',(16.7670277653193,18.2851235392682,-22.));
#115584=CARTESIAN_POINT('Ctrl Pts',(16.7762620345021,18.2693657448798,-22.));
#115585=CARTESIAN_POINT('Ctrl Pts',(16.7856937256623,18.2537253744878,-22.));
#115586=CARTESIAN_POINT('Ctrl Pts',(16.7953227326228,18.2382075784408,-22.));
#115587=CARTESIAN_POINT('Ctrl Pts',(16.8035476401832,18.2249525835537,-22.));
#115588=CARTESIAN_POINT('Ctrl Pts',(16.8119142470167,18.2117907879613,-22.));
#115589=CARTESIAN_POINT('Ctrl Pts',(16.8204179429878,18.198731704156,-22.));
#115590=CARTESIAN_POINT('Ctrl Pts',(16.8615694556779,18.1355355298381,-22.));
#115591=CARTESIAN_POINT('Ctrl Pts',(16.9059580849723,18.0746943089279,-22.));
#115592=CARTESIAN_POINT('Ctrl Pts',(16.9535504550157,18.0165477730385,-22.));
#115593=CARTESIAN_POINT('Ctrl Pts',(16.9976827241168,17.9626286560281,-22.));
#115594=CARTESIAN_POINT('Ctrl Pts',(17.0445703727031,17.9110265261487,-22.));
#115595=CARTESIAN_POINT('Ctrl Pts',(17.0942093579555,17.8620454496849,-22.));
#115596=CARTESIAN_POINT('Ctrl Pts',(17.0997979190133,17.8565309587036,-22.));
#115597=CARTESIAN_POINT('Ctrl Pts',(17.1054213743828,17.8510497281848,-22.));
#115598=CARTESIAN_POINT('Ctrl Pts',(17.1110793555412,17.8456019071633,-22.));
#115599=CARTESIAN_POINT('Ctrl Pts',(20.3539256943887,-20.3149122292573,
-22.));
#115600=CARTESIAN_POINT('Ctrl Pts',(20.408139566195,-20.2625995855167,-22.));
#115601=CARTESIAN_POINT('Ctrl Pts',(20.4591341972937,-20.2073573541925,
-22.));
#115602=CARTESIAN_POINT('Ctrl Pts',(20.5069159265706,-20.1495677196682,
-22.));
#115603=CARTESIAN_POINT('Ctrl Pts',(20.5546976558475,-20.091778085144,-22.));
#115604=CARTESIAN_POINT('Ctrl Pts',(20.5992668013762,-20.0314403792713,
-22.));
#115605=CARTESIAN_POINT('Ctrl Pts',(20.6406036312651,-19.9688911346062,
-22.));
#115606=CARTESIAN_POINT('Ctrl Pts',(20.6814854208042,-19.9070304388754,
-22.));
#115607=CARTESIAN_POINT('Ctrl Pts',(20.7192059247084,-19.8430059080155,
-22.));
#115608=CARTESIAN_POINT('Ctrl Pts',(20.7537163516506,-19.7771088559497,
-22.));
#115609=CARTESIAN_POINT('Ctrl Pts',(20.7688146634378,-19.748278895671,-22.));
#115610=CARTESIAN_POINT('Ctrl Pts',(20.7832981375853,-19.7190901423257,
-22.));
#115611=CARTESIAN_POINT('Ctrl Pts',(20.7971606745034,-19.6895654320343,
-22.));
#115612=CARTESIAN_POINT('Ctrl Pts',(20.8039890054239,-19.6750223153312,
-22.));
#115613=CARTESIAN_POINT('Ctrl Pts',(20.8106666589183,-19.660397672949,-22.));
#115614=CARTESIAN_POINT('Ctrl Pts',(20.8171927881263,-19.6456941670648,
-22.));
#115615=CARTESIAN_POINT('Ctrl Pts',(20.8232049803476,-19.6321485719831,
-22.));
#115616=CARTESIAN_POINT('Ctrl Pts',(20.8290890410869,-19.618534653263,-22.));
#115617=CARTESIAN_POINT('Ctrl Pts',(20.8348363668121,-19.6048740328408,
-22.));
#115618=CARTESIAN_POINT('Ctrl Pts',(20.8661434568434,-19.5304612896112,
-22.));
#115619=CARTESIAN_POINT('Ctrl Pts',(20.8934547915536,-19.4545373140852,
-21.9999999999999));
#115620=CARTESIAN_POINT('Ctrl Pts',(20.916748098317,-19.3774919314298,-22.));
#115621=CARTESIAN_POINT('Ctrl Pts',(20.9400414050804,-19.3004465487744,
-22.));
#115622=CARTESIAN_POINT('Ctrl Pts',(20.9593170648394,-19.2222788660794,
-21.9999999999999));
#115623=CARTESIAN_POINT('Ctrl Pts',(20.9745132363111,-19.1433443390627,
-21.9999999999999));
#115624=CARTESIAN_POINT('Ctrl Pts',(20.9885143247977,-19.0706175144489,
-21.9999999999999));
#115625=CARTESIAN_POINT('Ctrl Pts',(20.9990521599664,-18.9972388060651,
-22.));
#115626=CARTESIAN_POINT('Ctrl Pts',(21.0060443782249,-18.923470317406,-22.));
#115627=CARTESIAN_POINT('Ctrl Pts',(21.0087022983456,-18.8954290373673,
-22.));
#115628=CARTESIAN_POINT('Ctrl Pts',(21.010847535719,-18.8673313285427,-22.));
#115629=CARTESIAN_POINT('Ctrl Pts',(21.012474202948,-18.8391913006101,-22.));
#115630=CARTESIAN_POINT('Ctrl Pts',(21.0133676804257,-18.8237348626051,
-22.));
#115631=CARTESIAN_POINT('Ctrl Pts',(21.0141046936245,-18.8082656553794,
-22.));
#115632=CARTESIAN_POINT('Ctrl Pts',(21.0146841647679,-18.7927860097385,
-22.));
#115633=CARTESIAN_POINT('Ctrl Pts',(21.0151318658524,-18.7808263906625,
-22.));
#115634=CARTESIAN_POINT('Ctrl Pts',(21.01548535769,-18.768863838497,-22.));
#115635=CARTESIAN_POINT('Ctrl Pts',(21.0157442193216,-18.7569079719692,
-22.));
#115636=CARTESIAN_POINT('Ctrl Pts',(21.017551069503,-18.6734562086591,-22.));
#115637=CARTESIAN_POINT('Ctrl Pts',(21.0147560903276,-18.5902106853063,
-22.));
#115638=CARTESIAN_POINT('Ctrl Pts',(21.0073030399704,-18.5075520380822,
-22.));
#115639=CARTESIAN_POINT('Ctrl Pts',(20.9998642034238,-18.4250510302545,
-22.));
#115640=CARTESIAN_POINT('Ctrl Pts',(20.9877854202568,-18.3431336582205,
-22.));
#115641=CARTESIAN_POINT('Ctrl Pts',(20.9709614068361,-18.2621627589815,
-22.));
#115642=CARTESIAN_POINT('Ctrl Pts',(20.9545236784523,-18.1830509789684,
-22.));
#115643=CARTESIAN_POINT('Ctrl Pts',(20.9335563404747,-18.104841755941,-22.));
#115644=CARTESIAN_POINT('Ctrl Pts',(20.9083250537327,-18.0277615701596,
-22.));
#115645=CARTESIAN_POINT('Ctrl Pts',(20.8979276440165,-17.9959980584227,
-22.));
#115646=CARTESIAN_POINT('Ctrl Pts',(20.8868055423579,-17.9644263425748,
-22.));
#115647=CARTESIAN_POINT('Ctrl Pts',(20.874974854388,-17.9330627463293,-22.));
#115648=CARTESIAN_POINT('Ctrl Pts',(20.8684235902148,-17.9156951000059,
-22.));
#115649=CARTESIAN_POINT('Ctrl Pts',(20.8616527986486,-17.8983861321004,
-22.));
#115650=CARTESIAN_POINT('Ctrl Pts',(20.854677607217,-17.8811686926409,-22.));
#115651=CARTESIAN_POINT('Ctrl Pts',(20.8226256793881,-17.8020522795121,
-22.));
#115652=CARTESIAN_POINT('Ctrl Pts',(20.7862268153504,-17.724765227739,-22.));
#115653=CARTESIAN_POINT('Ctrl Pts',(20.7458439642001,-17.6495556859564,
-22.));
#115654=CARTESIAN_POINT('Ctrl Pts',(20.7054483430734,-17.5743223612055,
-22.));
#115655=CARTESIAN_POINT('Ctrl Pts',(20.6610656710241,-17.501167065488,-22.));
#115656=CARTESIAN_POINT('Ctrl Pts',(20.6130013967575,-17.4303438070485,
-22.));
#115657=CARTESIAN_POINT('Ctrl Pts',(20.5649371224908,-17.359520548609,-22.));
#115658=CARTESIAN_POINT('Ctrl Pts',(20.5131906957729,-17.2910285130232,
-22.));
#115659=CARTESIAN_POINT('Ctrl Pts',(20.4580179345364,-17.2251393904043,
-22.));
#115660=CARTESIAN_POINT('Ctrl Pts',(20.4361042290218,-17.1989693239199,
-22.));
#115661=CARTESIAN_POINT('Ctrl Pts',(20.4136494990236,-17.1732101420222,
-22.));
#115662=CARTESIAN_POINT('Ctrl Pts',(20.3906678986206,-17.1478800862692,
-22.));
#115663=CARTESIAN_POINT('Ctrl Pts',(20.3815361507949,-17.1378151788001,
-22.));
#115664=CARTESIAN_POINT('Ctrl Pts',(20.3723204509639,-17.1278172287239,
-22.));
#115665=CARTESIAN_POINT('Ctrl Pts',(20.3630239943621,-17.1178899237497,
-22.));
#115666=CARTESIAN_POINT('Ctrl Pts',(20.3025144308281,-17.0532742409372,
-22.));
#115667=CARTESIAN_POINT('Ctrl Pts',(20.2387850776616,-16.9918596463668,
-22.));
#115668=CARTESIAN_POINT('Ctrl Pts',(20.1721440203356,-16.9339205021469,
-22.));
#115669=CARTESIAN_POINT('Ctrl Pts',(20.1169511671352,-16.8859346686413,
-22.));
#115670=CARTESIAN_POINT('Ctrl Pts',(20.0597599562651,-16.8403327947037,
-22.));
#115671=CARTESIAN_POINT('Ctrl Pts',(20.0007222507865,-16.7972847116374,
-22.));
#115672=CARTESIAN_POINT('Ctrl Pts',(19.9812253134723,-16.7830682753746,
-22.));
#115673=CARTESIAN_POINT('Ctrl Pts',(19.9615268410592,-16.7691304877775,
-22.));
#115674=CARTESIAN_POINT('Ctrl Pts',(19.94163187493,-16.7554778736493,-22.));
#115675=CARTESIAN_POINT('Ctrl Pts',(19.9257068621322,-16.7445495788584,
-22.));
#115676=CARTESIAN_POINT('Ctrl Pts',(19.9096545851051,-16.733803248942,-22.));
#115677=CARTESIAN_POINT('Ctrl Pts',(19.8934935740057,-16.7232524113246,
-22.));
#115678=CARTESIAN_POINT('Ctrl Pts',(19.818965815021,-16.6745964034672,-22.));
#115679=CARTESIAN_POINT('Ctrl Pts',(19.7420559170313,-16.630044080676,-22.));
#115680=CARTESIAN_POINT('Ctrl Pts',(19.6630447444111,-16.5898860460099,
-22.));
#115681=CARTESIAN_POINT('Ctrl Pts',(19.585203529837,-16.5503226514967,-22.));
#115682=CARTESIAN_POINT('Ctrl Pts',(19.5053221290521,-16.5150236485074,
-22.));
#115683=CARTESIAN_POINT('Ctrl Pts',(19.4236366733768,-16.4843042822826,
-22.));
#115684=CARTESIAN_POINT('Ctrl Pts',(19.4149419062245,-16.481034450044,-22.));
#115685=CARTESIAN_POINT('Ctrl Pts',(19.4062266741651,-16.4778165460524,
-22.));
#115686=CARTESIAN_POINT('Ctrl Pts',(19.3974913926779,-16.4746504400725,
-22.));
#115687=CARTESIAN_POINT('Ctrl Pts',(18.0722627314314,-16.4790050975816,
-22.));
#115688=CARTESIAN_POINT('Ctrl Pts',(17.9909906838445,-16.5084318215279,
-22.));
#115689=CARTESIAN_POINT('Ctrl Pts',(17.9115928093154,-16.5422181704993,
-22.));
#115690=CARTESIAN_POINT('Ctrl Pts',(17.8342682750801,-16.580050621616,-22.));
#115691=CARTESIAN_POINT('Ctrl Pts',(17.7547379110741,-16.6189623155343,
-22.));
#115692=CARTESIAN_POINT('Ctrl Pts',(17.6774001286652,-16.6621548599534,
-22.));
#115693=CARTESIAN_POINT('Ctrl Pts',(17.6025009734493,-16.7093334978469,
-22.));
#115694=CARTESIAN_POINT('Ctrl Pts',(17.5320732406115,-16.7536956070808,
-22.));
#115695=CARTESIAN_POINT('Ctrl Pts',(17.463801490032,-16.8015830463496,-22.));
#115696=CARTESIAN_POINT('Ctrl Pts',(17.3979216159377,-16.8527787647009,
-22.));
#115697=CARTESIAN_POINT('Ctrl Pts',(17.368253233471,-16.875834275562,-22.));
#115698=CARTESIAN_POINT('Ctrl Pts',(17.3390703919806,-16.89956103538,-22.));
#115699=CARTESIAN_POINT('Ctrl Pts',(17.3103970329429,-16.9239405076492,
-22.));
#115700=CARTESIAN_POINT('Ctrl Pts',(17.2926918239748,-16.938994329927,-22.));
#115701=CARTESIAN_POINT('Ctrl Pts',(17.2751809015629,-16.9542970328152,
-22.));
#115702=CARTESIAN_POINT('Ctrl Pts',(17.257870215766,-16.9698443651112,-22.));
#115703=CARTESIAN_POINT('Ctrl Pts',(17.2457081778958,-16.9807675166481,
-22.));
#115704=CARTESIAN_POINT('Ctrl Pts',(17.2336432038411,-16.9918132192483,
-22.));
#115705=CARTESIAN_POINT('Ctrl Pts',(17.2216942554371,-17.0029639093079,
-22.));
#115706=CARTESIAN_POINT('Ctrl Pts',(17.1582584279828,-17.0621618593448,
-22.));
#115707=CARTESIAN_POINT('Ctrl Pts',(17.0979853415004,-17.1244075418475,
-22.));
#115708=CARTESIAN_POINT('Ctrl Pts',(17.0411056012962,-17.1894227118676,
-22.));
#115709=CARTESIAN_POINT('Ctrl Pts',(16.9845622276309,-17.2540534053124,
-22.));
#115710=CARTESIAN_POINT('Ctrl Pts',(16.9313716721992,-17.321421754448,-22.));
#115711=CARTESIAN_POINT('Ctrl Pts',(16.8818040511554,-17.3912811759233,
-22.));
#115712=CARTESIAN_POINT('Ctrl Pts',(16.8334273398594,-17.4594621576379,
-22.));
#115713=CARTESIAN_POINT('Ctrl Pts',(16.7885012591507,-17.5300167108658,
-22.));
#115714=CARTESIAN_POINT('Ctrl Pts',(16.7473243285991,-17.6027294194541,
-22.));
#115715=CARTESIAN_POINT('Ctrl Pts',(16.7339893719969,-17.6262770904551,
-22.));
#115716=CARTESIAN_POINT('Ctrl Pts',(16.7210480077419,-17.6500511631478,
-22.));
#115717=CARTESIAN_POINT('Ctrl Pts',(16.7085115583106,-17.6740444448892,
-22.));
#115718=CARTESIAN_POINT('Ctrl Pts',(16.6986548564673,-17.6929090066348,
-22.));
#115719=CARTESIAN_POINT('Ctrl Pts',(16.6890484758239,-17.7119090799142,
-22.));
#115720=CARTESIAN_POINT('Ctrl Pts',(16.679698188427,-17.7310411708259,-22.));
#115721=CARTESIAN_POINT('Ctrl Pts',(16.6737722417175,-17.7431665469103,
-22.));
#115722=CARTESIAN_POINT('Ctrl Pts',(16.6679529881854,-17.7553371759649,
-22.));
#115723=CARTESIAN_POINT('Ctrl Pts',(16.6622430964078,-17.7675484960222,
-22.));
#115724=CARTESIAN_POINT('Ctrl Pts',(16.6271175593077,-17.8426688647472,
-22.));
#115725=CARTESIAN_POINT('Ctrl Pts',(16.5961054609041,-17.9193709825623,
-22.));
#115726=CARTESIAN_POINT('Ctrl Pts',(16.5694535992104,-17.9974262815892,
-22.));
#115727=CARTESIAN_POINT('Ctrl Pts',(16.5428017375166,-18.0754815806163,
-22.));
#115728=CARTESIAN_POINT('Ctrl Pts',(16.5205096404242,-18.1548907906356,
-22.));
#115729=CARTESIAN_POINT('Ctrl Pts',(16.502878414596,-18.2354346063206,-22.));
#115730=CARTESIAN_POINT('Ctrl Pts',(16.4850539457493,-18.3168612040769,
-22.));
#115731=CARTESIAN_POINT('Ctrl Pts',(16.4719938146952,-18.3994486405796,
-22.));
#115732=CARTESIAN_POINT('Ctrl Pts',(16.4636223620895,-18.4828054643466,
-22.));
#115733=CARTESIAN_POINT('Ctrl Pts',(16.4601638961884,-18.5172423471919,
-22.));
#115734=CARTESIAN_POINT('Ctrl Pts',(16.4575062577843,-18.5518103876793,
-22.));
#115735=CARTESIAN_POINT('Ctrl Pts',(16.455646533733,-18.5864810569274,-22.));
#115736=CARTESIAN_POINT('Ctrl Pts',(16.4549145761463,-18.6001268767863,
-22.));
#115737=CARTESIAN_POINT('Ctrl Pts',(16.4543062363129,-18.6137905856188,
-22.));
#115738=CARTESIAN_POINT('Ctrl Pts',(16.4538218073552,-18.6274527865309,
-22.));
#115739=CARTESIAN_POINT('Ctrl Pts',(16.4509320250045,-18.7089524294446,
-22.));
#115740=CARTESIAN_POINT('Ctrl Pts',(16.4524388232547,-18.790528997647,-22.));
#115741=CARTESIAN_POINT('Ctrl Pts',(16.4582089280278,-18.8718234286525,
-22.));
#115742=CARTESIAN_POINT('Ctrl Pts',(16.4640073807546,-18.9535172511518,
-22.));
#115743=CARTESIAN_POINT('Ctrl Pts',(16.4741115013324,-19.034927191256,-22.));
#115744=CARTESIAN_POINT('Ctrl Pts',(16.4884372995143,-19.1156771272516,
-22.));
#115745=CARTESIAN_POINT('Ctrl Pts',(16.5025241468048,-19.1950801736051,
-22.));
#115746=CARTESIAN_POINT('Ctrl Pts',(16.52069350435,-19.2738459251496,-22.));
#115747=CARTESIAN_POINT('Ctrl Pts',(16.5429083122977,-19.3515913790962,
-22.));
#115748=CARTESIAN_POINT('Ctrl Pts',(16.5522119453725,-19.3841514254605,
-22.));
#115749=CARTESIAN_POINT('Ctrl Pts',(16.5622256148023,-19.416532131398,-22.));
#115750=CARTESIAN_POINT('Ctrl Pts',(16.5729485780652,-19.4487034546206,
-22.));
#115751=CARTESIAN_POINT('Ctrl Pts',(16.578489253474,-19.4653267382297,-22.));
#115752=CARTESIAN_POINT('Ctrl Pts',(16.5842201861179,-19.481896150472,-22.));
#115753=CARTESIAN_POINT('Ctrl Pts',(16.5901333903942,-19.4983861799902,
-22.));
#115754=CARTESIAN_POINT('Ctrl Pts',(16.6168665612538,-19.5729364163756,
-22.));
#115755=CARTESIAN_POINT('Ctrl Pts',(16.6473526072598,-19.6459624977086,
-22.));
#115756=CARTESIAN_POINT('Ctrl Pts',(16.6815326752298,-19.7171051627545,
-22.));
#115757=CARTESIAN_POINT('Ctrl Pts',(16.7078448962084,-19.7718716285595,
-22.));
#115758=CARTESIAN_POINT('Ctrl Pts',(16.7363471421602,-19.8255215876092,
-22.));
#115759=CARTESIAN_POINT('Ctrl Pts',(16.7670277670848,-19.8778764601534,
-22.));
#115760=CARTESIAN_POINT('Ctrl Pts',(16.7762620361372,-19.8936342545421,
-22.));
#115761=CARTESIAN_POINT('Ctrl Pts',(16.7856937271573,-19.9092746249327,
-22.));
#115762=CARTESIAN_POINT('Ctrl Pts',(16.7953227339677,-19.9247924209762,
-22.));
#115763=CARTESIAN_POINT('Ctrl Pts',(16.8035476416632,-19.9380474162847,
-21.9999999999999));
#115764=CARTESIAN_POINT('Ctrl Pts',(16.8119142486341,-19.9512092122917,
-22.));
#115765=CARTESIAN_POINT('Ctrl Pts',(16.8204179447442,-19.9642682965029,
-22.));
#115766=CARTESIAN_POINT('Ctrl Pts',(16.8615694572081,-20.0274644714052,
-22.));
#115767=CARTESIAN_POINT('Ctrl Pts',(16.905958086176,-20.0883056928111,-21.9999999999999));
#115768=CARTESIAN_POINT('Ctrl Pts',(16.9535504557831,-20.1464522290647,
-22.));
#115769=CARTESIAN_POINT('Ctrl Pts',(16.9976827257099,-20.2003713479159,
-22.));
#115770=CARTESIAN_POINT('Ctrl Pts',(17.0445703751811,-20.251973479394,-22.));
#115771=CARTESIAN_POINT('Ctrl Pts',(17.0942093613684,-20.3009545571532,
-22.));
#115772=CARTESIAN_POINT('Ctrl Pts',(17.0997979224383,-20.3064690481884,
-22.));
#115773=CARTESIAN_POINT('Ctrl Pts',(17.1054213778192,-20.3119502787582,
-22.));
#115774=CARTESIAN_POINT('Ctrl Pts',(17.1110793589886,-20.3173980998282,
-22.));
#115775=CARTESIAN_POINT('Ctrl Pts',(-17.1140743056112,-20.3149122292573,
-22.));
#115776=CARTESIAN_POINT('Ctrl Pts',(-17.0603910881415,-20.2631116303188,
-22.));
#115777=CARTESIAN_POINT('Ctrl Pts',(-17.009864429043,-20.2084384430965,
-22.));
#115778=CARTESIAN_POINT('Ctrl Pts',(-16.9624880608118,-20.1512639730765,
-22.));
#115779=CARTESIAN_POINT('Ctrl Pts',(-16.9134243877873,-20.0920532398113,
-22.));
#115780=CARTESIAN_POINT('Ctrl Pts',(-16.867738891267,-20.0301594501991,
-22.));
#115781=CARTESIAN_POINT('Ctrl Pts',(-16.8254529492616,-19.9659454033071,
-22.));
#115782=CARTESIAN_POINT('Ctrl Pts',(-16.7853184507726,-19.904998468091,
-22.));
#115783=CARTESIAN_POINT('Ctrl Pts',(-16.7482463250022,-19.8419604355298,
-22.));
#115784=CARTESIAN_POINT('Ctrl Pts',(-16.71428331717,-19.777108745806,-22.));
#115785=CARTESIAN_POINT('Ctrl Pts',(-16.6991849978544,-19.7482788045816,
-22.));
#115786=CARTESIAN_POINT('Ctrl Pts',(-16.6847015153359,-19.7190900711551,
-22.));
#115787=CARTESIAN_POINT('Ctrl Pts',(-16.6708389693358,-19.6895653814969,
-22.));
#115788=CARTESIAN_POINT('Ctrl Pts',(-16.6640105788719,-19.6750221576682,
-22.));
#115789=CARTESIAN_POINT('Ctrl Pts',(-16.6573328680918,-19.6603974070189,
-22.));
#115790=CARTESIAN_POINT('Ctrl Pts',(-16.6508066838924,-19.6456937917726,
-22.));
#115791=CARTESIAN_POINT('Ctrl Pts',(-16.6447945515434,-19.6321483449743,
-22.));
#115792=CARTESIAN_POINT('Ctrl Pts',(-16.6389105480172,-19.6185345763602,
-22.));
#115793=CARTESIAN_POINT('Ctrl Pts',(-16.6331632765825,-19.6048741071589,
-22.));
#115794=CARTESIAN_POINT('Ctrl Pts',(-16.6018561398417,-19.530461373728,
-22.));
#115795=CARTESIAN_POINT('Ctrl Pts',(-16.5745447598008,-19.4545374092054,
-22.));
#115796=CARTESIAN_POINT('Ctrl Pts',(-16.5512514111518,-19.3774920371772,
-22.));
#115797=CARTESIAN_POINT('Ctrl Pts',(-16.5279580625028,-19.3004466651491,
-22.));
#115798=CARTESIAN_POINT('Ctrl Pts',(-16.5086823642981,-19.2222789927081,
-22.));
#115799=CARTESIAN_POINT('Ctrl Pts',(-16.4934861598923,-19.1433444740215,
-22.));
#115800=CARTESIAN_POINT('Ctrl Pts',(-16.4781825851218,-19.0638522352736,
-22.));
#115801=CARTESIAN_POINT('Ctrl Pts',(-16.4670158957966,-18.9835813665502,
-22.));
#115802=CARTESIAN_POINT('Ctrl Pts',(-16.4600957863878,-18.9028735673802,
-22.));
#115803=CARTESIAN_POINT('Ctrl Pts',(-16.4582781144994,-18.8816744375601,
-22.));
#115804=CARTESIAN_POINT('Ctrl Pts',(-16.4567536954935,-18.8604450906499,
-22.));
#115805=CARTESIAN_POINT('Ctrl Pts',(-16.4555251072067,-18.8391916010845,
-22.));
#115806=CARTESIAN_POINT('Ctrl Pts',(-16.4546315989448,-18.8237346992684,
-22.));
#115807=CARTESIAN_POINT('Ctrl Pts',(-16.45389456466,-18.8082650273129,-22.));
#115808=CARTESIAN_POINT('Ctrl Pts',(-16.4533150822428,-18.7927849162226,
-22.));
#115809=CARTESIAN_POINT('Ctrl Pts',(-16.4528673708036,-18.7808248936061,
-22.));
#115810=CARTESIAN_POINT('Ctrl Pts',(-16.4525138752178,-18.7688619391664,
-22.));
#115811=CARTESIAN_POINT('Ctrl Pts',(-16.4522550163972,-18.7569056703414,
-22.));
#115812=CARTESIAN_POINT('Ctrl Pts',(-16.4504482477209,-18.6734539573408,
-22.));
#115813=CARTESIAN_POINT('Ctrl Pts',(-16.4532433131771,-18.5902084834056,
-22.));
#115814=CARTESIAN_POINT('Ctrl Pts',(-16.4606964571555,-18.5075498822213,
-22.));
#115815=CARTESIAN_POINT('Ctrl Pts',(-16.4681352990784,-18.4250498970387,
-22.));
#115816=CARTESIAN_POINT('Ctrl Pts',(-16.4802139851741,-18.3431335304585,
-22.));
#115817=CARTESIAN_POINT('Ctrl Pts',(-16.4970377976341,-18.2621636043343,
-22.));
#115818=CARTESIAN_POINT('Ctrl Pts',(-16.5135061122501,-18.1829046241824,
-22.));
#115819=CARTESIAN_POINT('Ctrl Pts',(-16.5345209017837,-18.1045515514237,
-22.));
#115820=CARTESIAN_POINT('Ctrl Pts',(-16.5598150664329,-18.027332141339,
-22.));
#115821=CARTESIAN_POINT('Ctrl Pts',(-16.5701720519776,-17.9957137690736,
-22.));
#115822=CARTESIAN_POINT('Ctrl Pts',(-16.5812471270599,-17.964285535797,
-22.));
#115823=CARTESIAN_POINT('Ctrl Pts',(-16.5930244062011,-17.9330635460661,
-22.));
#115824=CARTESIAN_POINT('Ctrl Pts',(-16.5995756745648,-17.9156958984863,
-22.));
#115825=CARTESIAN_POINT('Ctrl Pts',(-16.606346470602,-17.8983869289424,
-22.));
#115826=CARTESIAN_POINT('Ctrl Pts',(-16.613321666761,-17.8811694874779,
-22.));
#115827=CARTESIAN_POINT('Ctrl Pts',(-16.6442808434086,-17.804750444978,
-22.));
#115828=CARTESIAN_POINT('Ctrl Pts',(-16.6792959255797,-17.7300381471314,
-22.));
#115829=CARTESIAN_POINT('Ctrl Pts',(-16.7180388949534,-17.6572562073793,
-22.));
#115830=CARTESIAN_POINT('Ctrl Pts',(-16.7588458333272,-17.5805969275616,
-22.));
#115831=CARTESIAN_POINT('Ctrl Pts',(-16.8037884744598,-17.5060783091779,
-22.));
#115832=CARTESIAN_POINT('Ctrl Pts',(-16.852544028446,-17.4339672739469,
-22.));
#115833=CARTESIAN_POINT('Ctrl Pts',(-16.9012995824321,-17.3618562387159,
-22.));
#115834=CARTESIAN_POINT('Ctrl Pts',(-16.9538686479157,-17.2921519008718,
-22.));
#115835=CARTESIAN_POINT('Ctrl Pts',(-17.0099816867116,-17.2251398785991,
-22.));
#115836=CARTESIAN_POINT('Ctrl Pts',(-17.0318954130067,-17.1989697914665,
-22.));
#115837=CARTESIAN_POINT('Ctrl Pts',(-17.0543501640382,-17.1732105886975,
-22.));
#115838=CARTESIAN_POINT('Ctrl Pts',(-17.0773317856131,-17.1478805119615,
-22.));
#115839=CARTESIAN_POINT('Ctrl Pts',(-17.0864635488618,-17.1378155884281,
-22.));
#115840=CARTESIAN_POINT('Ctrl Pts',(-17.095679264258,-17.127817622382,-22.));
#115841=CARTESIAN_POINT('Ctrl Pts',(-17.1049757365821,-17.1178903015161,
-22.));
#115842=CARTESIAN_POINT('Ctrl Pts',(-17.165485351815,-17.0532745693386,
-22.));
#115843=CARTESIAN_POINT('Ctrl Pts',(-17.2292147565865,-16.9918599247989,
-22.));
#115844=CARTESIAN_POINT('Ctrl Pts',(-17.2958558635168,-16.9339207318737,
-22.));
#115845=CARTESIAN_POINT('Ctrl Pts',(-17.3510487599444,-16.8859348561654,
-22.));
#115846=CARTESIAN_POINT('Ctrl Pts',(-17.4082400128264,-16.8403329410748,
-22.));
#115847=CARTESIAN_POINT('Ctrl Pts',(-17.4672777580111,-16.7972848189689,
-22.));
#115848=CARTESIAN_POINT('Ctrl Pts',(-17.4896865553589,-16.7809451596297,
-22.));
#115849=CARTESIAN_POINT('Ctrl Pts',(-17.5123617016702,-16.7649735008075,
-22.));
#115850=CARTESIAN_POINT('Ctrl Pts',(-17.5352952134256,-16.7493800153535,
-22.));
#115851=CARTESIAN_POINT('Ctrl Pts',(-17.5482870635507,-16.7405462951581,
-22.));
#115852=CARTESIAN_POINT('Ctrl Pts',(-17.561360861439,-16.7318346842869,
-22.));
#115853=CARTESIAN_POINT('Ctrl Pts',(-17.5745065855726,-16.7232523975405,
-22.));
#115854=CARTESIAN_POINT('Ctrl Pts',(-17.6490343908001,-16.674596348734,
-22.));
#115855=CARTESIAN_POINT('Ctrl Pts',(-17.7259443303905,-16.6300439893022,
-22.));
#115856=CARTESIAN_POINT('Ctrl Pts',(-17.8049555380688,-16.5898859241833,
-22.));
#115857=CARTESIAN_POINT('Ctrl Pts',(-17.8827967752859,-16.5503225057145,
-22.));
#115858=CARTESIAN_POINT('Ctrl Pts',(-17.962678191744,-16.51502348347,-22.));
#115859=CARTESIAN_POINT('Ctrl Pts',(-18.0443636543755,-16.484304104371,
-22.));
#115860=CARTESIAN_POINT('Ctrl Pts',(-18.0530584200154,-16.4810342716093,
-22.));
#115861=CARTESIAN_POINT('Ctrl Pts',(-18.0617736504531,-16.47781636714,-22.));
#115862=CARTESIAN_POINT('Ctrl Pts',(-18.0705089302108,-16.4746502607264,
-22.));
#115863=CARTESIAN_POINT('Ctrl Pts',(-19.3957372685685,-16.4790050975816,
-22.));
#115864=CARTESIAN_POINT('Ctrl Pts',(-19.4773890957418,-16.5085693309101,
-22.));
#115865=CARTESIAN_POINT('Ctrl Pts',(-19.5571492106161,-16.5425339973349,
-22.));
#115866=CARTESIAN_POINT('Ctrl Pts',(-19.6348155858968,-16.5805812675105,
-22.));
#115867=CARTESIAN_POINT('Ctrl Pts',(-19.7143272387952,-16.6195325038595,
-22.));
#115868=CARTESIAN_POINT('Ctrl Pts',(-19.7916452000862,-16.662763296461,
-22.));
#115869=CARTESIAN_POINT('Ctrl Pts',(-19.8665232562821,-16.7099790585762,
-22.));
#115870=CARTESIAN_POINT('Ctrl Pts',(-19.9365886725381,-16.754160120352,
-22.));
#115871=CARTESIAN_POINT('Ctrl Pts',(-20.0045178827344,-16.8018313324451,
-22.));
#115872=CARTESIAN_POINT('Ctrl Pts',(-20.0700783280693,-16.8527788406207,
-22.));
#115873=CARTESIAN_POINT('Ctrl Pts',(-20.0997467181299,-16.8758343665167,
-22.));
#115874=CARTESIAN_POINT('Ctrl Pts',(-20.1289295668893,-16.8995611421252,
-22.));
#115875=CARTESIAN_POINT('Ctrl Pts',(-20.1576029328649,-16.9239406308391,
-22.));
#115876=CARTESIAN_POINT('Ctrl Pts',(-20.1753081453826,-16.9389944626467,
-22.));
#115877=CARTESIAN_POINT('Ctrl Pts',(-20.1928190712341,-16.9542971752936,
-22.));
#115878=CARTESIAN_POINT('Ctrl Pts',(-20.2101297603596,-16.9698445175537,
-22.));
#115879=CARTESIAN_POINT('Ctrl Pts',(-20.2222917967556,-16.9807676726665,
-22.));
#115880=CARTESIAN_POINT('Ctrl Pts',(-20.2343567693431,-16.9918133788689,
-22.));
#115881=CARTESIAN_POINT('Ctrl Pts',(-20.2463057162916,-17.002964072546,
-22.));
#115882=CARTESIAN_POINT('Ctrl Pts',(-20.3097375002003,-17.0621582755838,
-22.));
#115883=CARTESIAN_POINT('Ctrl Pts',(-20.3700069454282,-17.1243998240975,
-22.));
#115884=CARTESIAN_POINT('Ctrl Pts',(-20.4268834922199,-17.1894105241984,
-22.));
#115885=CARTESIAN_POINT('Ctrl Pts',(-20.483037632838,-17.2535955037914,
-22.));
#115886=CARTESIAN_POINT('Ctrl Pts',(-20.535884967494,-17.3204805753055,
-22.));
#115887=CARTESIAN_POINT('Ctrl Pts',(-20.585161092451,-17.389824149674,-22.));
#115888=CARTESIAN_POINT('Ctrl Pts',(-20.6305983299564,-17.4537654693455,
-22.));
#115889=CARTESIAN_POINT('Ctrl Pts',(-20.6729989843627,-17.519797868898,
-22.));
#115890=CARTESIAN_POINT('Ctrl Pts',(-20.7121180645734,-17.5877431573068,
-22.));
#115891=CARTESIAN_POINT('Ctrl Pts',(-20.7391058385126,-17.6346177789475,
-22.));
#115892=CARTESIAN_POINT('Ctrl Pts',(-20.7645310103452,-17.6824030516845,
-22.));
#115893=CARTESIAN_POINT('Ctrl Pts',(-20.788301742955,-17.7310415486134,
-22.0000000000001));
#115894=CARTESIAN_POINT('Ctrl Pts',(-20.7942276911041,-17.7431669305097,
-22.0000000000001));
#115895=CARTESIAN_POINT('Ctrl Pts',(-20.8000469460378,-17.755337565341,
-22.));
#115896=CARTESIAN_POINT('Ctrl Pts',(-20.8057568391674,-17.7675488911101,
-22.));
#115897=CARTESIAN_POINT('Ctrl Pts',(-20.8408823751017,-17.8426692746921,
-22.));
#115898=CARTESIAN_POINT('Ctrl Pts',(-20.8718944728201,-17.9193714043448,
-22.));
#115899=CARTESIAN_POINT('Ctrl Pts',(-20.8985463344755,-17.9974267111826,
-22.));
#115900=CARTESIAN_POINT('Ctrl Pts',(-20.9251981961308,-18.0754820180205,
-22.));
#115901=CARTESIAN_POINT('Ctrl Pts',(-20.9474902938315,-18.1548912318264,
-22.));
#115902=CARTESIAN_POINT('Ctrl Pts',(-20.9651215210881,-18.2354350462128,
-22.));
#115903=CARTESIAN_POINT('Ctrl Pts',(-20.9829459910005,-18.3168616409281,
-22.));
#115904=CARTESIAN_POINT('Ctrl Pts',(-20.9960061241615,-18.3994490691394,
-22.));
#115905=CARTESIAN_POINT('Ctrl Pts',(-21.0043775797276,-18.4828058803714,
-22.));
#115906=CARTESIAN_POINT('Ctrl Pts',(-21.007836047032,-18.5172427598331,
-22.));
#115907=CARTESIAN_POINT('Ctrl Pts',(-21.0104936869016,-18.5518107962264,
-22.));
#115908=CARTESIAN_POINT('Ctrl Pts',(-21.012353412468,-18.5864814607357,
-22.));
#115909=CARTESIAN_POINT('Ctrl Pts',(-21.0130853706128,-18.6001272780164,
-22.));
#115910=CARTESIAN_POINT('Ctrl Pts',(-21.013693711025,-18.613790984168,-22.));
#115911=CARTESIAN_POINT('Ctrl Pts',(-21.0141781405805,-18.627453182305,
-22.));
#115912=CARTESIAN_POINT('Ctrl Pts',(-21.0170629011428,-18.7088110803349,
-22.));
#115913=CARTESIAN_POINT('Ctrl Pts',(-21.0155663446046,-18.7902456314198,
-22.));
#115914=CARTESIAN_POINT('Ctrl Pts',(-21.0098210964673,-18.8713996487605,
-22.));
#115915=CARTESIAN_POINT('Ctrl Pts',(-21.0040551877191,-18.9528455058144,
-22.));
#115916=CARTESIAN_POINT('Ctrl Pts',(-20.9940096006471,-19.0340098255527,
-22.));
#115917=CARTESIAN_POINT('Ctrl Pts',(-20.9797677148279,-19.1145199798923,
-22.));
#115918=CARTESIAN_POINT('Ctrl Pts',(-20.9656475419196,-19.1943420845335,
-22.));
#115919=CARTESIAN_POINT('Ctrl Pts',(-20.9474020500876,-19.2735220803043,
-22.));
#115920=CARTESIAN_POINT('Ctrl Pts',(-20.9250689726277,-19.3516710302886,
-22.));
#115921=CARTESIAN_POINT('Ctrl Pts',(-20.9157717541756,-19.3842042922679,
-22.));
#115922=CARTESIAN_POINT('Ctrl Pts',(-20.9057656547729,-19.4165584812898,
-22.));
#115923=CARTESIAN_POINT('Ctrl Pts',(-20.8950514146661,-19.4487036278629,
-22.));
#115924=CARTESIAN_POINT('Ctrl Pts',(-20.8895107411906,-19.4653269029819,
-22.));
#115925=CARTESIAN_POINT('Ctrl Pts',(-20.8837798105413,-19.4818963067406,
-22.));
#115926=CARTESIAN_POINT('Ctrl Pts',(-20.8778666083137,-19.4983863278128,
-22.));
#115927=CARTESIAN_POINT('Ctrl Pts',(-20.8511334402601,-19.5729365440179,
-22.));
#115928=CARTESIAN_POINT('Ctrl Pts',(-20.8206473963514,-19.6459626051823,
-22.));
#115929=CARTESIAN_POINT('Ctrl Pts',(-20.7864673296103,-19.7171052508947,
-22.));
#115930=CARTESIAN_POINT('Ctrl Pts',(-20.7601551154116,-19.771871689674,
-22.));
#115931=CARTESIAN_POINT('Ctrl Pts',(-20.7316528766953,-19.8255216226873,
-22.));
#115932=CARTESIAN_POINT('Ctrl Pts',(-20.7009722593753,-19.8778764706885,
-22.));
#115933=CARTESIAN_POINT('Ctrl Pts',(-20.691737989898,-19.893634262321,-22.));
#115934=CARTESIAN_POINT('Ctrl Pts',(-20.6823062983705,-19.9092746300216,
-22.));
#115935=CARTESIAN_POINT('Ctrl Pts',(-20.6726772909679,-19.9247924234514,
-22.));
#115936=CARTESIAN_POINT('Ctrl Pts',(-20.6644523795805,-19.9380474216617,
-22.));
#115937=CARTESIAN_POINT('Ctrl Pts',(-20.6560857687532,-19.9512092205436,
-22.));
#115938=CARTESIAN_POINT('Ctrl Pts',(-20.6475820686168,-19.9642683076145,
-22.));
#115939=CARTESIAN_POINT('Ctrl Pts',(-20.6064305516755,-20.0274644733087,
-22.));
#115940=CARTESIAN_POINT('Ctrl Pts',(-20.5620419166416,-20.0883056868182,
-22.));
#115941=CARTESIAN_POINT('Ctrl Pts',(-20.5144495392311,-20.1464522171397,
-22.));
#115942=CARTESIAN_POINT('Ctrl Pts',(-20.4703172870207,-20.2003713000042,
-22.));
#115943=CARTESIAN_POINT('Ctrl Pts',(-20.4234296568856,-20.2519733998006,
-22.));
#115944=CARTESIAN_POINT('Ctrl Pts',(-20.3737906915119,-20.3009544512441,
-22.));
#115945=CARTESIAN_POINT('Ctrl Pts',(-20.368202130628,-20.3064689414452,
-22.));
#115946=CARTESIAN_POINT('Ctrl Pts',(-20.3625786754248,-20.3119501712233,
-22.));
#115947=CARTESIAN_POINT('Ctrl Pts',(-20.3569206944252,-20.3173979915434,
-22.));
#115948=CARTESIAN_POINT('Ctrl Pts',(-23.5308805332535,12.9159404490031,
-3.78088374166161));
#115949=CARTESIAN_POINT('Ctrl Pts',(-23.4920947707073,12.3929457330403,
-3.32818299800387));
#115950=CARTESIAN_POINT('Ctrl Pts',(-23.414527126525,11.1227145575666,-2.68291372642237));
#115951=CARTESIAN_POINT('Ctrl Pts',(-23.2981776007066,8.98517233796921,
-2.72051551203619));
#115952=CARTESIAN_POINT('Ctrl Pts',(-23.1818319557984,7.11449327439195,
-3.75456823383891));
#115953=CARTESIAN_POINT('Ctrl Pts',(-23.0654863108902,5.94567083410245,
-5.54430593302147));
#115954=CARTESIAN_POINT('Ctrl Pts',(-22.949140665982,5.75110708678027,-7.67299084799178));
#115955=CARTESIAN_POINT('Ctrl Pts',(-22.8327950210738,6.57598682635251,
-9.64497510434418));
#115956=CARTESIAN_POINT('Ctrl Pts',(-22.7164493761656,8.22829836165371,
-11.0010927381981));
#115957=CARTESIAN_POINT('Ctrl Pts',(-22.6001037312574,10.3232843871488,
-11.4255808825339));
#115958=CARTESIAN_POINT('Ctrl Pts',(-22.4837580863492,12.373152711629,-10.8195997802356));
#115959=CARTESIAN_POINT('Ctrl Pts',(-22.367412441441,13.9005991739366,-9.32424845126734));
#115960=CARTESIAN_POINT('Ctrl Pts',(-22.2510667965328,14.5499677602782,
-7.28771036251242));
#115961=CARTESIAN_POINT('Ctrl Pts',(-22.1347211516246,14.1700608207003,
-5.18418037574749));
#115962=CARTESIAN_POINT('Ctrl Pts',(-22.0183755067164,12.8493270829512,
-3.5034534546303));
#115963=CARTESIAN_POINT('Ctrl Pts',(-21.9020298618082,10.8953137792879,
-2.63687434737169));
#115964=CARTESIAN_POINT('Ctrl Pts',(-21.7856842169001,8.76295316144695,
-2.78622511569276));
#115965=CARTESIAN_POINT('Ctrl Pts',(-21.6693385719918,6.94885218972505,
-3.91672099675241));
#115966=CARTESIAN_POINT('Ctrl Pts',(-21.5529929270836,5.87520384764723,
-5.7651525900255));
#115967=CARTESIAN_POINT('Ctrl Pts',(-21.4366472821754,5.79243819862009,
-7.90108306247407));
#115968=CARTESIAN_POINT('Ctrl Pts',(-21.3203016372673,6.71891118246527,
-9.82725987337206));
#115969=CARTESIAN_POINT('Ctrl Pts',(-21.2039559923591,8.44081429108934,
-11.0950054485607));
#115970=CARTESIAN_POINT('Ctrl Pts',(-21.0876103474509,10.5532071885089,
-11.4095079136007));
#115971=CARTESIAN_POINT('Ctrl Pts',(-20.9712647025427,12.5726070805758,
-10.6967524773169));
#115972=CARTESIAN_POINT('Ctrl Pts',(-20.8549190576345,14.01129149844,-9.12434942623869));
#115973=CARTESIAN_POINT('Ctrl Pts',(-20.6997915310902,14.7563922376921,
-6.36488911986088));
#115974=CARTESIAN_POINT('Ctrl Pts',(-20.5058821229099,12.994051845457,-2.90538039035574));
#115975=CARTESIAN_POINT('Ctrl Pts',(-20.2731908330935,8.33355232269001,
-2.33672443840605));
#115976=CARTESIAN_POINT('Ctrl Pts',(-20.0792814249132,5.79107032299367,
-5.27097555050355));
#115977=CARTESIAN_POINT('Ctrl Pts',(-19.9241538983689,5.85079178660098,
-8.12863711914554));
#115978=CARTESIAN_POINT('Ctrl Pts',(-19.8078082534607,6.86917854738371,
-10.0008424002799));
#115979=CARTESIAN_POINT('Ctrl Pts',(-19.6914626085525,8.65794742930395,
-11.1782557190028));
#115980=CARTESIAN_POINT('Ctrl Pts',(-19.5751169636443,10.7839875685715,
-11.3809103015019));
#115981=CARTESIAN_POINT('Ctrl Pts',(-19.4587713187361,12.7602040696624,
-10.5643948394832));
#115982=CARTESIAN_POINT('Ctrl Pts',(-19.3424256738279,14.1226489554401,
-8.91750284853353));
#115983=CARTESIAN_POINT('Ctrl Pts',(-19.2260800289197,14.5559010795726,
-6.82433736708493));
#115984=CARTESIAN_POINT('Ctrl Pts',(-19.1097343840116,13.9582122926688,
-4.77197574410858));
#115985=CARTESIAN_POINT('Ctrl Pts',(-18.9933887391034,12.4691657270705,
-3.23844269973861));
#115986=CARTESIAN_POINT('Ctrl Pts',(-18.8770430941952,10.4352783026865,
-2.58074261501136));
#115987=CARTESIAN_POINT('Ctrl Pts',(-18.760697449287,8.33022292180678,-2.95205001253969));
#115988=CARTESIAN_POINT('Ctrl Pts',(-18.6443518043788,6.64410352432277,
-4.2658924562235));
#115989=CARTESIAN_POINT('Ctrl Pts',(-18.5280061594706,5.76954396207305,
-6.21635733927994));
#115990=CARTESIAN_POINT('Ctrl Pts',(-18.4116605145624,5.91017031183124,
-8.34928752511129));
#115991=CARTESIAN_POINT('Ctrl Pts',(-18.2953148696542,7.0332421902222,-10.1680447514146));
#115992=CARTESIAN_POINT('Ctrl Pts',(-18.178969224746,8.87725972928098,-11.2491426006833));
#115993=CARTESIAN_POINT('Ctrl Pts',(-18.0626235798378,11.0128500131701,
-11.3408528567028));
#115994=CARTESIAN_POINT('Ctrl Pts',(-17.9462779349296,12.9427659614882,
-10.4218246313654));
#115995=CARTESIAN_POINT('Ctrl Pts',(-17.8299322900214,14.2176127610098,
-8.70604080762527));
#115996=CARTESIAN_POINT('Ctrl Pts',(-17.7135866451132,14.5406046262916,
-6.59302619008096));
#115997=CARTESIAN_POINT('Ctrl Pts',(-17.597241000205,13.8364209745585,-4.57475160186675));
#115998=CARTESIAN_POINT('Ctrl Pts',(-17.4808953552968,12.2692662804362,
-3.12122783010914));
#115999=CARTESIAN_POINT('Ctrl Pts',(-17.3645497103886,10.2035478774237,
-2.57077055143018));
#116000=CARTESIAN_POINT('Ctrl Pts',(-17.2869859471165,8.81549756936472,
-2.89162768514917));
#116001=CARTESIAN_POINT('Ctrl Pts',(-17.2482040654804,8.19904022858213,
-3.20522926485876));
#116002=CARTESIAN_POINT('Ctrl Pts',(-23.6934851051207,13.100263928033,-3.56793868900448));
#116003=CARTESIAN_POINT('Ctrl Pts',(-23.6546993425745,12.5426730283998,
-3.08529171912816));
#116004=CARTESIAN_POINT('Ctrl Pts',(-23.5771316983922,11.1884158585721,
-2.39733778256787));
#116005=CARTESIAN_POINT('Ctrl Pts',(-23.4607821725738,8.90947488106098,
-2.43742693228256));
#116006=CARTESIAN_POINT('Ctrl Pts',(-23.3444365276657,6.91505009979918,
-3.53988240615246));
#116007=CARTESIAN_POINT('Ctrl Pts',(-23.2280908827574,5.66890986912247,
-5.4480115388869));
#116008=CARTESIAN_POINT('Ctrl Pts',(-23.1117452378493,5.46147569895942,
-7.71750929966068));
#116009=CARTESIAN_POINT('Ctrl Pts',(-22.9953995929411,6.34092136454444,
-9.81994062831756));
#116010=CARTESIAN_POINT('Ctrl Pts',(-22.8790539480329,8.10253357079198,
-11.265765659412));
#116011=CARTESIAN_POINT('Ctrl Pts',(-22.7627083031247,10.3361032551902,
-11.7183337620325));
#116012=CARTESIAN_POINT('Ctrl Pts',(-22.6463626582165,12.5215706954729,
-11.0722669134044));
#116013=CARTESIAN_POINT('Ctrl Pts',(-22.5300170133083,14.1500579842821,
-9.47799785611141));
#116014=CARTESIAN_POINT('Ctrl Pts',(-22.4136713684001,14.8423824059262,
-7.30674244876793));
#116015=CARTESIAN_POINT('Ctrl Pts',(-22.2973257234919,14.4373445618512,
-5.06406361870253));
#116016=CARTESIAN_POINT('Ctrl Pts',(-22.1809800785837,13.0292440772185,
-3.27215634434632));
#116017=CARTESIAN_POINT('Ctrl Pts',(-22.0646344336755,10.9459724826303,
-2.34825289126802));
#116018=CARTESIAN_POINT('Ctrl Pts',(-21.9482887887673,8.67255587065623,
-2.50748323667555));
#116019=CARTESIAN_POINT('Ctrl Pts',(-21.8319431438591,6.73845183102772,
-3.71276160013153));
#116020=CARTESIAN_POINT('Ctrl Pts',(-21.7155974989509,5.59378148030178,
-5.68346723738891));
#116021=CARTESIAN_POINT('Ctrl Pts',(-21.5992518540427,5.50554087042331,
-7.96068985042091));
#116022=CARTESIAN_POINT('Ctrl Pts',(-21.4829062091345,6.49330018955362,
-10.0142835638186));
#116023=CARTESIAN_POINT('Ctrl Pts',(-21.3665605642263,8.32910746277151,
-11.3658907105068));
#116024=CARTESIAN_POINT('Ctrl Pts',(-21.2502149193181,10.5812354864414,
-11.7011975636472));
#116025=CARTESIAN_POINT('Ctrl Pts',(-21.1338692744099,12.7342190026592,
-10.9412932418523));
#116026=CARTESIAN_POINT('Ctrl Pts',(-21.0175236295017,14.2680726236628,
-9.26487547877277));
#116027=CARTESIAN_POINT('Ctrl Pts',(-20.8623961029575,15.0624618953634,
-6.32287643409223));
#116028=CARTESIAN_POINT('Ctrl Pts',(-20.6684866947772,13.1835424057901,
-2.63452065171533));
#116029=CARTESIAN_POINT('Ctrl Pts',(-20.4357954049608,8.21475009809699,
-2.02824801806984));
#116030=CARTESIAN_POINT('Ctrl Pts',(-20.2418859967804,5.50408250960656,
-5.15660030807799));
#116031=CARTESIAN_POINT('Ctrl Pts',(-20.0867584702362,5.56775455753331,
-8.20329664414551));
#116032=CARTESIAN_POINT('Ctrl Pts',(-19.970412825328,6.65350776456926,-10.1993486024987));
#116033=CARTESIAN_POINT('Ctrl Pts',(-19.8540671804198,8.56060399262535,
-11.4546479995839));
#116034=CARTESIAN_POINT('Ctrl Pts',(-19.7377215355116,10.8272820253628,
-11.6707082149582));
#116035=CARTESIAN_POINT('Ctrl Pts',(-19.6213758906034,12.9342255624209,
-10.8001801252177));
#116036=CARTESIAN_POINT('Ctrl Pts',(-19.5050302456952,14.3867963941607,
-9.04434596704268));
#116037=CARTESIAN_POINT('Ctrl Pts',(-19.388684600787,14.8487082152359,-6.8127172559693));
#116038=CARTESIAN_POINT('Ctrl Pts',(-19.2723389558788,14.211482219985,-4.62459158509811));
#116039=CARTESIAN_POINT('Ctrl Pts',(-19.1559933109706,12.6239349871618,
-2.98961508585478));
#116040=CARTESIAN_POINT('Ctrl Pts',(-19.0396476660624,10.4555055860592,
-2.28840803588138));
#116041=CARTESIAN_POINT('Ctrl Pts',(-18.9233020211542,8.2112004568156,-2.68427747683199));
#116042=CARTESIAN_POINT('Ctrl Pts',(-18.8069563762461,6.41354399292294,
-4.08503080720052));
#116043=CARTESIAN_POINT('Ctrl Pts',(-18.6906107313378,5.48113217648616,
-6.16451925259414));
#116044=CARTESIAN_POINT('Ctrl Pts',(-18.5742650864296,5.6310609816548,-8.43854310957185));
#116045=CARTESIAN_POINT('Ctrl Pts',(-18.4579194415215,6.82842424348439,
-10.3776114157632));
#116046=CARTESIAN_POINT('Ctrl Pts',(-18.3415737966133,8.79442383613891,
-11.5302240597658));
#116047=CARTESIAN_POINT('Ctrl Pts',(-18.2252281517051,11.0712837570842,
-11.6280009638123));
#116048=CARTESIAN_POINT('Ctrl Pts',(-18.1088825067969,13.128863952437,-10.6481788751495));
#116049=CARTESIAN_POINT('Ctrl Pts',(-17.9925368618887,14.4880420705777,
-8.8188956784843));
#116050=CARTESIAN_POINT('Ctrl Pts',(-17.8761912169805,14.8323998991367,
-6.56610480780444));
#116051=CARTESIAN_POINT('Ctrl Pts',(-17.7598455720723,14.0816343868042,
-4.4143210344682));
#116052=CARTESIAN_POINT('Ctrl Pts',(-17.6434999271641,12.4108121603283,
-2.86464643395019));
#116053=CARTESIAN_POINT('Ctrl Pts',(-17.5271542822559,10.2084461562965,
-2.27777631870772));
#116054=CARTESIAN_POINT('Ctrl Pts',(-17.4495905189838,8.72857609951769,
-2.61985820287125));
#116055=CARTESIAN_POINT('Ctrl Pts',(-17.4108086373477,8.07134000756269,
-2.9542045769733));
#116056=CARTESIAN_POINT('Ctrl Pts',(-23.856089676988,13.284587407063,-3.35499363634734));
#116057=CARTESIAN_POINT('Ctrl Pts',(-23.8173039144417,12.6924003237593,
-2.84240044025244));
#116058=CARTESIAN_POINT('Ctrl Pts',(-23.7397362702595,11.2541171595776,
-2.11176183871335));
#116059=CARTESIAN_POINT('Ctrl Pts',(-23.6233867444411,8.83377742415274,
-2.15433835252893));
#116060=CARTESIAN_POINT('Ctrl Pts',(-23.5070410995329,6.7156069252064,-3.325196578466));
#116061=CARTESIAN_POINT('Ctrl Pts',(-23.3906954546247,5.39214890414247,
-5.35171714475233));
#116062=CARTESIAN_POINT('Ctrl Pts',(-23.2743498097165,5.17184431113857,
-7.76202775132957));
#116063=CARTESIAN_POINT('Ctrl Pts',(-23.1580041648084,6.10585590273637,
-9.99490615229094));
#116064=CARTESIAN_POINT('Ctrl Pts',(-23.0416585199001,7.97676877993027,
-11.530438580626));
#116065=CARTESIAN_POINT('Ctrl Pts',(-22.925312874992,10.3489221232315,-12.0110866415312));
#116066=CARTESIAN_POINT('Ctrl Pts',(-22.8089672300837,12.669988679317,-11.3249340465732));
#116067=CARTESIAN_POINT('Ctrl Pts',(-22.6926215851756,14.3995167946276,
-9.63174726095547));
#116068=CARTESIAN_POINT('Ctrl Pts',(-22.5762759402673,15.1347970515741,
-7.32577453502343));
#116069=CARTESIAN_POINT('Ctrl Pts',(-22.4599302953592,14.7046283030022,
-4.94394686165757));
#116070=CARTESIAN_POINT('Ctrl Pts',(-22.343584650451,13.2091610714859,-3.04085923406232));
#116071=CARTESIAN_POINT('Ctrl Pts',(-22.2272390055428,10.9966311859728,
-2.05963143516434));
#116072=CARTESIAN_POINT('Ctrl Pts',(-22.1108933606346,8.58215857986552,
-2.22874135765833));
#116073=CARTESIAN_POINT('Ctrl Pts',(-21.9945477157264,6.5280514723304,-3.50880220351063));
#116074=CARTESIAN_POINT('Ctrl Pts',(-21.8782020708182,5.31235911295633,
-5.60178188475233));
#116075=CARTESIAN_POINT('Ctrl Pts',(-21.76185642591,5.21864354222653,-8.02029663836774));
#116076=CARTESIAN_POINT('Ctrl Pts',(-21.6455107810018,6.26768919664197,
-10.201307254265));
#116077=CARTESIAN_POINT('Ctrl Pts',(-21.5291651360936,8.21740063445369,
-11.6367759724529));
#116078=CARTESIAN_POINT('Ctrl Pts',(-21.4128194911854,10.609263784374,-11.9928872136937));
#116079=CARTESIAN_POINT('Ctrl Pts',(-21.2964738462772,12.8958309247427,
-11.1858340063878));
#116080=CARTESIAN_POINT('Ctrl Pts',(-21.180128201369,14.5248537488857,-9.40540153130685));
#116081=CARTESIAN_POINT('Ctrl Pts',(-21.0250006748248,15.3685315530349,
-6.28086374832358));
#116082=CARTESIAN_POINT('Ctrl Pts',(-20.8310912666444,13.3730329661233,
-2.36366091307492));
#116083=CARTESIAN_POINT('Ctrl Pts',(-20.598399976828,8.09594787350394,-1.71977159773362));
#116084=CARTESIAN_POINT('Ctrl Pts',(-20.4044905686477,5.21709469621947,
-5.04222506565243));
#116085=CARTESIAN_POINT('Ctrl Pts',(-20.2493630421035,5.28471732846564,
-8.27795616914549));
#116086=CARTESIAN_POINT('Ctrl Pts',(-20.1330173971953,6.43783698175481,
-10.3978548047174));
#116087=CARTESIAN_POINT('Ctrl Pts',(-20.0166717522871,8.46326055594674,
-11.7310402801651));
#116088=CARTESIAN_POINT('Ctrl Pts',(-19.9003261073789,10.8705764821541,
-11.9605061284144));
#116089=CARTESIAN_POINT('Ctrl Pts',(-19.7839804624707,13.1082470551796,
-11.0359654109521));
#116090=CARTESIAN_POINT('Ctrl Pts',(-19.6676348175625,14.6509438328813,
-9.17118908555184));
#116091=CARTESIAN_POINT('Ctrl Pts',(-19.5512891726543,15.1415153508992,
-6.80109714485368));
#116092=CARTESIAN_POINT('Ctrl Pts',(-19.4349435277461,14.464752147301,-4.47720742608763));
#116093=CARTESIAN_POINT('Ctrl Pts',(-19.3185978828379,12.7787042472532,
-2.74078747197094));
#116094=CARTESIAN_POINT('Ctrl Pts',(-19.2022522379297,10.4757328694319,
-1.9960734567514));
#116095=CARTESIAN_POINT('Ctrl Pts',(-19.0859065930215,8.09217799182441,
-2.41650494112427));
#116096=CARTESIAN_POINT('Ctrl Pts',(-18.9695609481133,6.18298446152309,
-3.90416915817754));
#116097=CARTESIAN_POINT('Ctrl Pts',(-18.8532153032051,5.19272039089927,
-6.11268116590833));
#116098=CARTESIAN_POINT('Ctrl Pts',(-18.7368696582969,5.35195165147837,
-8.52779869403239));
#116099=CARTESIAN_POINT('Ctrl Pts',(-18.6205240133887,6.62360629674656,
-10.5871780801117));
#116100=CARTESIAN_POINT('Ctrl Pts',(-18.5041783684805,8.71158794299683,
-11.8113055188485));
#116101=CARTESIAN_POINT('Ctrl Pts',(-18.3878327235723,11.1297175009982,
-11.9151490709219));
#116102=CARTESIAN_POINT('Ctrl Pts',(-18.2714870786641,13.3149619433859,
-10.8745331189337));
#116103=CARTESIAN_POINT('Ctrl Pts',(-18.155141433756,14.7584713801457,-8.93175054934334));
#116104=CARTESIAN_POINT('Ctrl Pts',(-18.0387957888477,15.1241951719818,
-6.53918342552792));
#116105=CARTESIAN_POINT('Ctrl Pts',(-17.9224501439396,14.3268477990501,
-4.25389046706965));
#116106=CARTESIAN_POINT('Ctrl Pts',(-17.8061044990314,12.5523580402204,
-2.60806503779124));
#116107=CARTESIAN_POINT('Ctrl Pts',(-17.6897588541232,10.2133444351692,
-1.98478208598528));
#116108=CARTESIAN_POINT('Ctrl Pts',(-17.612195090851,8.64165462967066,-2.34808872059334));
#116109=CARTESIAN_POINT('Ctrl Pts',(-17.573413209215,7.94363978654326,-2.70317988908784));
#116110=CARTESIAN_POINT('Ctrl Pts',(-24.0186942488553,13.4689108860931,
-3.1420485836902));
#116111=CARTESIAN_POINT('Ctrl Pts',(-23.979908486309,12.8421276191188,-2.59950916137671));
#116112=CARTESIAN_POINT('Ctrl Pts',(-23.9023408421268,11.3198184605831,
-1.82618589485885));
#116113=CARTESIAN_POINT('Ctrl Pts',(-23.7859913163084,8.75807996724451,
-1.8712497727753));
#116114=CARTESIAN_POINT('Ctrl Pts',(-23.6696456714002,6.51616375061362,
-3.11051075077954));
#116115=CARTESIAN_POINT('Ctrl Pts',(-23.553300026492,5.11538793916249,-5.25542275061777));
#116116=CARTESIAN_POINT('Ctrl Pts',(-23.4369543815838,4.88221292331772,
-7.80654620299846));
#116117=CARTESIAN_POINT('Ctrl Pts',(-23.3206087366756,5.8707904409283,-10.1698716762644));
#116118=CARTESIAN_POINT('Ctrl Pts',(-23.2042630917674,7.85100398906855,
-11.7951115018399));
#116119=CARTESIAN_POINT('Ctrl Pts',(-23.0879174468592,10.3617409912729,
-12.3038395210299));
#116120=CARTESIAN_POINT('Ctrl Pts',(-22.971571801951,12.818406663161,-11.5776011797419));
#116121=CARTESIAN_POINT('Ctrl Pts',(-22.8552261570428,14.6489756049733,
-9.78549666579953));
#116122=CARTESIAN_POINT('Ctrl Pts',(-22.7388805121346,15.4272116972221,
-7.34480662127895));
#116123=CARTESIAN_POINT('Ctrl Pts',(-22.6225348672265,14.971912044153,-4.82383010461261));
#116124=CARTESIAN_POINT('Ctrl Pts',(-22.5061892223183,13.3890780657532,
-2.80956212377835));
#116125=CARTESIAN_POINT('Ctrl Pts',(-22.38984357741,11.0472898893152,-1.77100997906067));
#116126=CARTESIAN_POINT('Ctrl Pts',(-22.2734979325019,8.49176128907481,
-1.94999947864112));
#116127=CARTESIAN_POINT('Ctrl Pts',(-22.1571522875937,6.31765111363307,
-3.30484280688975));
#116128=CARTESIAN_POINT('Ctrl Pts',(-22.0408066426855,5.03093674561089,
-5.52009653211574));
#116129=CARTESIAN_POINT('Ctrl Pts',(-21.9244609977773,4.93174621402975,
-8.07990342631457));
#116130=CARTESIAN_POINT('Ctrl Pts',(-21.8081153528691,6.04207820373032,
-10.3883309447114));
#116131=CARTESIAN_POINT('Ctrl Pts',(-21.6917697079609,8.10569380613587,
-11.907661234399));
#116132=CARTESIAN_POINT('Ctrl Pts',(-21.5754240630527,10.6372920823065,
-12.2845768637402));
#116133=CARTESIAN_POINT('Ctrl Pts',(-21.4590784181445,13.0574428468262,
-11.4303747709233));
#116134=CARTESIAN_POINT('Ctrl Pts',(-21.3427327732363,14.7816348741085,
-9.54592758384092));
#116135=CARTESIAN_POINT('Ctrl Pts',(-21.187605246692,15.6746012107064,-6.23885106255491));
#116136=CARTESIAN_POINT('Ctrl Pts',(-20.9936958385117,13.5625235264562,
-2.09280117443452));
#116137=CARTESIAN_POINT('Ctrl Pts',(-20.7610045486953,7.97714564891089,
-1.41129517739739));
#116138=CARTESIAN_POINT('Ctrl Pts',(-20.567095140515,4.93010688283236,-4.9278498232269));
#116139=CARTESIAN_POINT('Ctrl Pts',(-20.4119676139707,5.00168009939798,
-8.35261569414545));
#116140=CARTESIAN_POINT('Ctrl Pts',(-20.2956219690625,6.22216619894035,
-10.5963610069362));
#116141=CARTESIAN_POINT('Ctrl Pts',(-20.1792763241544,8.36591711926816,
-12.0074325607462));
#116142=CARTESIAN_POINT('Ctrl Pts',(-20.0629306792461,10.9138709389455,
-12.2503040418707));
#116143=CARTESIAN_POINT('Ctrl Pts',(-19.946585034338,13.2822685479382,-11.2717506966864));
#116144=CARTESIAN_POINT('Ctrl Pts',(-19.8302393894298,14.915091271602,-9.298032204061));
#116145=CARTESIAN_POINT('Ctrl Pts',(-19.7138937445216,15.4343224865625,
-6.78947703373806));
#116146=CARTESIAN_POINT('Ctrl Pts',(-19.5975480996134,14.7180220746172,
-4.32982326707715));
#116147=CARTESIAN_POINT('Ctrl Pts',(-19.4812024547052,12.9334735073446,
-2.49195985808711));
#116148=CARTESIAN_POINT('Ctrl Pts',(-19.364856809797,10.4959601528046,-1.70373887762141));
#116149=CARTESIAN_POINT('Ctrl Pts',(-19.2485111648888,7.97315552683322,
-2.14873240541657));
#116150=CARTESIAN_POINT('Ctrl Pts',(-19.1321655199806,5.95242493012327,
-3.72330750915457));
#116151=CARTESIAN_POINT('Ctrl Pts',(-19.0158198750724,4.90430860531238,
-6.06084307922253));
#116152=CARTESIAN_POINT('Ctrl Pts',(-18.8994742301642,5.07284232130192,
-8.61705427849294));
#116153=CARTESIAN_POINT('Ctrl Pts',(-18.783128585256,6.41878835000875,-10.7967447444602));
#116154=CARTESIAN_POINT('Ctrl Pts',(-18.6667829403478,8.62875204985474,
-12.092386977931));
#116155=CARTESIAN_POINT('Ctrl Pts',(-18.5504372954396,11.1881512449122,
-12.2022971780315));
#116156=CARTESIAN_POINT('Ctrl Pts',(-18.4340916505314,13.5010599343348,
-11.1008873627179));
#116157=CARTESIAN_POINT('Ctrl Pts',(-18.3177460056232,15.0289006897138,
-9.04460542020237));
#116158=CARTESIAN_POINT('Ctrl Pts',(-18.201400360715,15.4159904448268,-6.5122620432514));
#116159=CARTESIAN_POINT('Ctrl Pts',(-18.0850547158068,14.572061211296,-4.0934598996711));
#116160=CARTESIAN_POINT('Ctrl Pts',(-17.9687090708987,12.6939039201125,
-2.35148364163229));
#116161=CARTESIAN_POINT('Ctrl Pts',(-17.8523634259905,10.218242714042,-1.69178785326283));
#116162=CARTESIAN_POINT('Ctrl Pts',(-17.7747996627183,8.55473315982364,
-2.07631923831543));
#116163=CARTESIAN_POINT('Ctrl Pts',(-17.7360177810823,7.81593956552383,
-2.45215520120238));
#116164=CARTESIAN_POINT('Ctrl Pts',(-17.734,7.81752421401937,-2.45527019889639));
#116165=CARTESIAN_POINT('Ctrl Pts',(-17.734,7.95501332932841,-2.39880616079668));
#116166=CARTESIAN_POINT('Ctrl Pts',(-17.734,8.09483307093979,-2.34855996252214));
#116167=CARTESIAN_POINT('Ctrl Pts',(-17.734,8.23654961332739,-2.304582486642));
#116168=CARTESIAN_POINT('Ctrl Pts',(-17.734,8.37832975988065,-2.26058527311788));
#116169=CARTESIAN_POINT('Ctrl Pts',(-17.734,8.52200921313304,-2.22286236353948));
#116170=CARTESIAN_POINT('Ctrl Pts',(-17.734,8.6671587240801,-2.19151622070739));
#116171=CARTESIAN_POINT('Ctrl Pts',(-17.734,8.73062405356116,-2.1778103992422));
#116172=CARTESIAN_POINT('Ctrl Pts',(-17.734,8.79437042286563,-2.16532435434159));
#116173=CARTESIAN_POINT('Ctrl Pts',(-17.734,8.85836166295589,-2.15406978045215));
#116174=CARTESIAN_POINT('Ctrl Pts',(-17.734,8.89040869116538,-2.1484334520045));
#116175=CARTESIAN_POINT('Ctrl Pts',(-17.734,8.92251712887926,-2.14310601138361));
#116176=CARTESIAN_POINT('Ctrl Pts',(-17.734,8.95468239459414,-2.13808910834503));
#116177=CARTESIAN_POINT('Ctrl Pts',(-17.734,8.98448154595258,-2.13344125452896));
#116178=CARTESIAN_POINT('Ctrl Pts',(-17.734,9.01432763175263,-2.12906034010219));
#116179=CARTESIAN_POINT('Ctrl Pts',(-17.734,9.04419731169371,-2.12495001478239));
#116180=CARTESIAN_POINT('Ctrl Pts',(-17.734,9.18914015305572,-2.10500463097011));
#116181=CARTESIAN_POINT('Ctrl Pts',(-17.734,9.33476318988617,-2.09140666587328));
#116182=CARTESIAN_POINT('Ctrl Pts',(-17.734,9.48065042336444,-2.08424512751231));
#116183=CARTESIAN_POINT('Ctrl Pts',(-17.734,9.62430709076033,-2.07719308663227));
#116184=CARTESIAN_POINT('Ctrl Pts',(-17.734,9.76822064380685,-2.07638225413068));
#116185=CARTESIAN_POINT('Ctrl Pts',(-17.734,9.91198516021645,-2.08194693812594));
#116186=CARTESIAN_POINT('Ctrl Pts',(-17.734,9.99104601795219,-2.08500714171915));
#116187=CARTESIAN_POINT('Ctrl Pts',(-17.734,10.0700615878024,-2.08999633223886));
#116188=CARTESIAN_POINT('Ctrl Pts',(-17.734,10.1489620547016,-2.09694320736949));
#116189=CARTESIAN_POINT('Ctrl Pts',(-17.734,10.1675473093435,-2.09857956578842));
#116190=CARTESIAN_POINT('Ctrl Pts',(-17.734,10.1861239058425,-2.10032440268515));
#116191=CARTESIAN_POINT('Ctrl Pts',(-17.734,10.204682003642,-2.10217705470482));
#116192=CARTESIAN_POINT('Ctrl Pts',(-17.734,10.2069686559161,-2.10240533084603));
#116193=CARTESIAN_POINT('Ctrl Pts',(-17.734,10.2092550663573,-2.10263524723068));
#116194=CARTESIAN_POINT('Ctrl Pts',(-17.734,10.2115412333789,-2.10286680408659));
#116195=CARTESIAN_POINT('Ctrl Pts',(-17.734,10.3540154766321,-2.11729745919824));
#116196=CARTESIAN_POINT('Ctrl Pts',(-17.734,10.4955450211138,-2.13809494422707));
#116197=CARTESIAN_POINT('Ctrl Pts',(-17.734,10.6357416460623,-2.16507440736953));
#116198=CARTESIAN_POINT('Ctrl Pts',(-17.734,10.7763962044387,-2.19214199530135));
#116199=CARTESIAN_POINT('Ctrl Pts',(-17.734,10.915709875811,-2.22543235084852));
#116200=CARTESIAN_POINT('Ctrl Pts',(-17.734,11.0532754223516,-2.26480926970525));
#116201=CARTESIAN_POINT('Ctrl Pts',(-17.734,11.1892331876652,-2.30372597543079));
#116202=CARTESIAN_POINT('Ctrl Pts',(-17.734,11.3234841068398,-2.34858822554395));
#116203=CARTESIAN_POINT('Ctrl Pts',(-17.734,11.4556098132251,-2.39930790770621));
#116204=CARTESIAN_POINT('Ctrl Pts',(-17.734,11.5858933052135,-2.44932041083996));
#116205=CARTESIAN_POINT('Ctrl Pts',(-17.734,11.7141110087283,-2.50502853561951));
#116206=CARTESIAN_POINT('Ctrl Pts',(-17.734,11.8398280865206,-2.56638422249516));
#116207=CARTESIAN_POINT('Ctrl Pts',(-17.734,11.8635810775125,-2.57797676905487));
#116208=CARTESIAN_POINT('Ctrl Pts',(-17.734,11.8872446880899,-2.58977102047971));
#116209=CARTESIAN_POINT('Ctrl Pts',(-17.734,11.9108158217838,-2.60176678408464));
#116210=CARTESIAN_POINT('Ctrl Pts',(-17.734,11.9371259496047,-2.61515646986953));
#116211=CARTESIAN_POINT('Ctrl Pts',(-17.734,11.9633250773611,-2.62879964621101));
#116212=CARTESIAN_POINT('Ctrl Pts',(-17.734,11.989373711485,-2.64267686049563));
#116213=CARTESIAN_POINT('Ctrl Pts',(-17.734,12.1092335086399,-2.7065312676527));
#116214=CARTESIAN_POINT('Ctrl Pts',(-17.734,12.2260636232258,-2.77541414480518));
#116215=CARTESIAN_POINT('Ctrl Pts',(-17.734,12.3395155043836,-2.84921040440292));
#116216=CARTESIAN_POINT('Ctrl Pts',(-17.734,12.3590922141296,-2.86194433124259));
#116217=CARTESIAN_POINT('Ctrl Pts',(-17.734,12.3785682723977,-2.87482464861868));
#116218=CARTESIAN_POINT('Ctrl Pts',(-17.734,12.397941804336,-2.88785087941439));
#116219=CARTESIAN_POINT('Ctrl Pts',(-17.734,12.5137183308796,-2.96569583614641));
#116220=CARTESIAN_POINT('Ctrl Pts',(-17.734,12.625836471894,-3.04874887784055));
#116221=CARTESIAN_POINT('Ctrl Pts',(-17.734,12.7340053685886,-3.13669684221413));
#116222=CARTESIAN_POINT('Ctrl Pts',(-17.734,12.8413651891065,-3.22398697790556));
#116223=CARTESIAN_POINT('Ctrl Pts',(-17.734,12.9448350524291,-3.31609977172436));
#116224=CARTESIAN_POINT('Ctrl Pts',(-17.734,13.0440889096059,-3.41275801808283));
#116225=CARTESIAN_POINT('Ctrl Pts',(-17.734,13.1288759097822,-3.49532773359962));
#116226=CARTESIAN_POINT('Ctrl Pts',(-17.734,13.2105858345264,-3.58121510518619));
#116227=CARTESIAN_POINT('Ctrl Pts',(-17.734,13.2889874920904,-3.67025872512399));
#116228=CARTESIAN_POINT('Ctrl Pts',(-17.734,13.3046808407887,-3.68808223320354));
#116229=CARTESIAN_POINT('Ctrl Pts',(-17.734,13.3202415499158,-3.70603222587404));
#116230=CARTESIAN_POINT('Ctrl Pts',(-17.734,13.3356676287495,-3.72410744241816));
#116231=CARTESIAN_POINT('Ctrl Pts',(-17.734,13.3480960124007,-3.73867016624531));
#116232=CARTESIAN_POINT('Ctrl Pts',(-17.734,13.3604375218648,-3.75331488553882));
#116233=CARTESIAN_POINT('Ctrl Pts',(-17.734,13.3726806466598,-3.76802811897179));
#116234=CARTESIAN_POINT('Ctrl Pts',(-17.734,13.4596595863362,-3.87255547327407));
#116235=CARTESIAN_POINT('Ctrl Pts',(-17.734,13.5418047089289,-3.98068713564629));
#116236=CARTESIAN_POINT('Ctrl Pts',(-17.734,13.6188521515589,-4.09212747512552));
#116237=CARTESIAN_POINT('Ctrl Pts',(-17.734,13.6955050681822,-4.20299717772693));
#116238=CARTESIAN_POINT('Ctrl Pts',(-17.734,13.7671127723516,-4.31714241929126));
#116239=CARTESIAN_POINT('Ctrl Pts',(-17.734,13.8333700251483,-4.43429573902715));
#116240=CARTESIAN_POINT('Ctrl Pts',(-17.734,13.8529952952312,-4.46899632566313));
#116241=CARTESIAN_POINT('Ctrl Pts',(-17.734,13.8721508267902,-4.50396094344829));
#116242=CARTESIAN_POINT('Ctrl Pts',(-17.734,13.89082783933,-4.53918291414616));
#116243=CARTESIAN_POINT('Ctrl Pts',(-17.734,13.9541037547201,-4.6585115505114));
#116244=CARTESIAN_POINT('Ctrl Pts',(-17.734,14.0118911506688,-4.78079380916986));
#116245=CARTESIAN_POINT('Ctrl Pts',(-17.734,14.0640355569298,-4.90562952893938));
#116246=CARTESIAN_POINT('Ctrl Pts',(-17.734,14.1069769502113,-5.00843288068094));
#116247=CARTESIAN_POINT('Ctrl Pts',(-17.734,14.1460905703569,-5.11296827640029));
#116248=CARTESIAN_POINT('Ctrl Pts',(-17.734,14.181263595494,-5.21901089821796));
#116249=CARTESIAN_POINT('Ctrl Pts',(-17.734,14.189228939926,-5.24302549474362));
#116250=CARTESIAN_POINT('Ctrl Pts',(-17.734,14.1969936498824,-5.26712264831227));
#116251=CARTESIAN_POINT('Ctrl Pts',(-17.734,14.2045469401604,-5.29126909440454));
#116252=CARTESIAN_POINT('Ctrl Pts',(-17.734,14.2441345445802,-5.41782320802469));
#116253=CARTESIAN_POINT('Ctrl Pts',(-17.734,14.2779661336648,-5.54586509835337));
#116254=CARTESIAN_POINT('Ctrl Pts',(-17.734,14.3059575691914,-5.67500275481729));
#116255=CARTESIAN_POINT('Ctrl Pts',(-17.734,14.3337111014893,-5.80304285180123));
#116256=CARTESIAN_POINT('Ctrl Pts',(-17.734,14.3557233452494,-5.93216096674691));
#116257=CARTESIAN_POINT('Ctrl Pts',(-17.734,14.3718618342398,-6.06197882817971));
#116258=CARTESIAN_POINT('Ctrl Pts',(-17.734,14.3878809810446,-6.19083670213723));
#116259=CARTESIAN_POINT('Ctrl Pts',(-17.734,14.3981129478511,-6.3203847452269));
#116260=CARTESIAN_POINT('Ctrl Pts',(-17.734,14.4023779577644,-6.45024544035567));
#116261=CARTESIAN_POINT('Ctrl Pts',(-17.734,14.404077015673,-6.50197822540308));
#116262=CARTESIAN_POINT('Ctrl Pts',(-17.734,14.4048285550272,-6.55376048351597));
#116263=CARTESIAN_POINT('Ctrl Pts',(-17.734,14.4046189505891,-6.60556761626202));
#116264=CARTESIAN_POINT('Ctrl Pts',(-17.734,14.4041999753073,-6.7091241450779));
#116265=CARTESIAN_POINT('Ctrl Pts',(-17.734,14.3999416905426,-6.8127807955209));
#116266=CARTESIAN_POINT('Ctrl Pts',(-17.734,14.3918515993157,-6.91632173312881));
#116267=CARTESIAN_POINT('Ctrl Pts',(-23.534,12.9193325810254,-3.77664721604209));
#116268=CARTESIAN_POINT('Ctrl Pts',(-23.534,12.8290342749467,-3.68176973928167));
#116269=CARTESIAN_POINT('Ctrl Pts',(-23.534,12.7344699653718,-3.59136003915295));
#116270=CARTESIAN_POINT('Ctrl Pts',(-23.534,12.6360835972834,-3.50554511160901));
#116271=CARTESIAN_POINT('Ctrl Pts',(-23.534,12.5375436323605,-3.41959621325707));
#116272=CARTESIAN_POINT('Ctrl Pts',(-23.534,12.4351690929809,-3.3382559634335));
#116273=CARTESIAN_POINT('Ctrl Pts',(-23.534,12.3293560803945,-3.26167549385162));
#116274=CARTESIAN_POINT('Ctrl Pts',(-23.534,12.2223961810545,-3.18426498338916));
#116275=CARTESIAN_POINT('Ctrl Pts',(-23.534,12.1119223277556,-3.11171743092941));
#116276=CARTESIAN_POINT('Ctrl Pts',(-23.534,11.9983009629288,-3.04422091350681));
#116277=CARTESIAN_POINT('Ctrl Pts',(-23.534,11.8876418446556,-2.97848411201814));
#116278=CARTESIAN_POINT('Ctrl Pts',(-23.534,11.7739964774381,-2.91753808376495));
#116279=CARTESIAN_POINT('Ctrl Pts',(-23.534,11.6576727871419,-2.86159294221042));
#116280=CARTESIAN_POINT('Ctrl Pts',(-23.534,11.6332495630019,-2.84984674736181));
#116281=CARTESIAN_POINT('Ctrl Pts',(-23.534,11.6087081820176,-2.83832114633447));
#116282=CARTESIAN_POINT('Ctrl Pts',(-23.534,11.5840513615887,-2.82701831535873));
#116283=CARTESIAN_POINT('Ctrl Pts',(-23.534,11.5622209636691,-2.81701113302431));
#116284=CARTESIAN_POINT('Ctrl Pts',(-23.534,11.5402959333441,-2.80717685242453));
#116285=CARTESIAN_POINT('Ctrl Pts',(-23.534,11.5183047885456,-2.79752845804063));
#116286=CARTESIAN_POINT('Ctrl Pts',(-23.534,11.3911942477278,-2.74175998216545));
#116287=CARTESIAN_POINT('Ctrl Pts',(-23.534,11.2617238431345,-2.69212530511711));
#116288=CARTESIAN_POINT('Ctrl Pts',(-23.534,11.1303326631264,-2.64879502193041));
#116289=CARTESIAN_POINT('Ctrl Pts',(-23.534,11.0033822809627,-2.60692922843141));
#116290=CARTESIAN_POINT('Ctrl Pts',(-23.534,10.8746380135545,-2.57094816886311));
#116291=CARTESIAN_POINT('Ctrl Pts',(-23.534,10.7445242523891,-2.54079174717233));
#116292=CARTESIAN_POINT('Ctrl Pts',(-23.534,10.6129949118633,-2.5103072371399));
#116293=CARTESIAN_POINT('Ctrl Pts',(-23.534,10.4800654160692,-2.48577456352108));
#116294=CARTESIAN_POINT('Ctrl Pts',(-23.534,10.3461486694481,-2.46717850660524));
#116295=CARTESIAN_POINT('Ctrl Pts',(-23.534,10.2117116901201,-2.44851020870933));
#116296=CARTESIAN_POINT('Ctrl Pts',(-23.534,10.0762789981111,-2.43582454855409));
#116297=CARTESIAN_POINT('Ctrl Pts',(-23.534,9.94025397651706,-2.4291562085726));
#116298=CARTESIAN_POINT('Ctrl Pts',(-23.534,9.92455348268286,-2.42838652495456));
#116299=CARTESIAN_POINT('Ctrl Pts',(-23.534,9.90884508947389,-2.42769706425968));
#116300=CARTESIAN_POINT('Ctrl Pts',(-23.534,9.89312941238514,-2.42708792441797));
#116301=CARTESIAN_POINT('Ctrl Pts',(-23.534,9.86982544152734,-2.42618466221429));
#116302=CARTESIAN_POINT('Ctrl Pts',(-23.534,9.84650207816375,-2.425458012161));
#116303=CARTESIAN_POINT('Ctrl Pts',(-23.534,9.82318746608169,-2.4249087042635));
#116304=CARTESIAN_POINT('Ctrl Pts',(-23.534,9.6848192673001,-2.42164865669821));
#116305=CARTESIAN_POINT('Ctrl Pts',(-23.534,9.54658084862224,-2.42462233472131));
#116306=CARTESIAN_POINT('Ctrl Pts',(-23.534,9.4089130640994,-2.43376529968541));
#116307=CARTESIAN_POINT('Ctrl Pts',(-23.534,9.26969699143324,-2.44301109149675));
#116308=CARTESIAN_POINT('Ctrl Pts',(-23.534,9.13106368650431,-2.45856549918628));
#116309=CARTESIAN_POINT('Ctrl Pts',(-23.534,8.99345056589427,-2.48041133999212));
#116310=CARTESIAN_POINT('Ctrl Pts',(-23.534,8.97031116329775,-2.48408467944715));
#116311=CARTESIAN_POINT('Ctrl Pts',(-23.534,8.94720057915598,-2.48793601825615));
#116312=CARTESIAN_POINT('Ctrl Pts',(-23.534,8.9241208670849,-2.49196541689415));
#116313=CARTESIAN_POINT('Ctrl Pts',(-23.534,8.7873871274078,-2.51583723742324));
#116314=CARTESIAN_POINT('Ctrl Pts',(-23.534,8.65173684163144,-2.54595438851017));
#116315=CARTESIAN_POINT('Ctrl Pts',(-23.534,8.51752579699817,-2.58210352084366));
#116316=CARTESIAN_POINT('Ctrl Pts',(-23.534,8.39200772104797,-2.61591124173702));
#116317=CARTESIAN_POINT('Ctrl Pts',(-23.534,8.2677479659076,-2.65499549928287));
#116318=CARTESIAN_POINT('Ctrl Pts',(-23.534,8.14504361020046,-2.69922256987843));
#116319=CARTESIAN_POINT('Ctrl Pts',(-23.534,8.12749669968016,-2.70554710861093));
#116320=CARTESIAN_POINT('Ctrl Pts',(-23.534,8.1099816141129,-2.71197687841997));
#116321=CARTESIAN_POINT('Ctrl Pts',(-23.534,8.09249924225049,-2.71851155118283));
#116322=CARTESIAN_POINT('Ctrl Pts',(-23.534,8.07453683564987,-2.72522565440019));
#116323=CARTESIAN_POINT('Ctrl Pts',(-23.534,8.05661738952652,-2.73204736696529));
#116324=CARTESIAN_POINT('Ctrl Pts',(-23.534,8.03874521119562,-2.73897465977803));
#116325=CARTESIAN_POINT('Ctrl Pts',(-23.534,7.90644077728776,-2.79025612850193));
#116326=CARTESIAN_POINT('Ctrl Pts',(-23.534,7.7766664785265,-2.84734176999563));
#116327=CARTESIAN_POINT('Ctrl Pts',(-23.534,7.64978171058123,-2.90995636965287));
#116328=CARTESIAN_POINT('Ctrl Pts',(-23.534,7.52165755880184,-2.97318257560338));
#116329=CARTESIAN_POINT('Ctrl Pts',(-23.534,7.3964789135714,-3.04204645157868));
#116330=CARTESIAN_POINT('Ctrl Pts',(-23.534,7.27461872474461,-3.11631789508779));
#116331=CARTESIAN_POINT('Ctrl Pts',(-23.534,7.1526351765545,-3.19066452375846));
#116332=CARTESIAN_POINT('Ctrl Pts',(-23.534,7.03397603466299,-3.27042992503056));
#116333=CARTESIAN_POINT('Ctrl Pts',(-23.534,6.91902974166616,-3.35543308861264));
#116334=CARTESIAN_POINT('Ctrl Pts',(-23.534,6.8844382354436,-3.3810136217932));
#116335=CARTESIAN_POINT('Ctrl Pts',(-23.534,6.85018311680615,-3.40706882775223));
#116336=CARTESIAN_POINT('Ctrl Pts',(-23.534,6.81627539023441,-3.43359460199418));
#116337=CARTESIAN_POINT('Ctrl Pts',(-23.534,6.76396915960913,-3.47451339559359));
#116338=CARTESIAN_POINT('Ctrl Pts',(-23.534,6.71248951985117,-3.51655187486384));
#116339=CARTESIAN_POINT('Ctrl Pts',(-23.534,6.66185982789805,-3.55967699429165));
#116340=CARTESIAN_POINT('Ctrl Pts',(-23.534,6.63093354887773,-3.58601923388978));
#116341=CARTESIAN_POINT('Ctrl Pts',(-23.534,6.60032442699024,-3.61276695671771));
#116342=CARTESIAN_POINT('Ctrl Pts',(-23.534,6.57003806517946,-3.63991298263474));
#116343=CARTESIAN_POINT('Ctrl Pts',(-23.534,6.54970174979597,-3.65814066372453));
#116344=CARTESIAN_POINT('Ctrl Pts',(-23.534,6.52950986024502,-3.67654895514717));
#116345=CARTESIAN_POINT('Ctrl Pts',(-23.534,6.50946759186945,-3.69513255143209));
#116346=CARTESIAN_POINT('Ctrl Pts',(-23.534,6.48629939547582,-3.71661457134924));
#116347=CARTESIAN_POINT('Ctrl Pts',(-23.534,6.46334194284684,-3.73832084889875));
#116348=CARTESIAN_POINT('Ctrl Pts',(-23.534,6.44060381946901,-3.76024083479514));
#116349=CARTESIAN_POINT('Ctrl Pts',(-23.534,6.33630358470948,-3.86078825627445));
#116350=CARTESIAN_POINT('Ctrl Pts',(-23.534,6.23656911791114,-3.96587231758902));
#116351=CARTESIAN_POINT('Ctrl Pts',(-23.534,6.14160415290407,-4.07509691447209));
#116352=CARTESIAN_POINT('Ctrl Pts',(-23.534,6.04554420161977,-4.18558091722884));
#116353=CARTESIAN_POINT('Ctrl Pts',(-23.5339999999999,5.95436378537622,
-4.30030196778979));
#116354=CARTESIAN_POINT('Ctrl Pts',(-23.534,5.86830289306953,-4.41889447743313));
#116355=CARTESIAN_POINT('Ctrl Pts',(-23.534,5.82757976366497,-4.47501123368759));
#116356=CARTESIAN_POINT('Ctrl Pts',(-23.534,5.788003413678,-4.53199543597994));
#116357=CARTESIAN_POINT('Ctrl Pts',(-23.534,5.74960209595384,-4.58981127009334));
#116358=CARTESIAN_POINT('Ctrl Pts',(-23.534,5.73602768423562,-4.61024848377764));
#116359=CARTESIAN_POINT('Ctrl Pts',(-23.534,5.72260309324962,-4.63078521650428));
#116360=CARTESIAN_POINT('Ctrl Pts',(-23.534,5.7093336961382,-4.65141296650499));
#116361=CARTESIAN_POINT('Ctrl Pts',(-23.534,5.62878693151663,-4.7766257783629));
#116362=CARTESIAN_POINT('Ctrl Pts',(-23.534,5.55390603885588,-4.90526364111016));
#116363=CARTESIAN_POINT('Ctrl Pts',(-23.534,5.48492211365497,-5.03693496093975));
#116364=CARTESIAN_POINT('Ctrl Pts',(-23.534,5.43386982584414,-5.13437972211843));
#116365=CARTESIAN_POINT('Ctrl Pts',(-23.534,5.38604780954608,-5.23348685196462));
#116366=CARTESIAN_POINT('Ctrl Pts',(-23.534,5.34156275575684,-5.33411058694693));
#116367=CARTESIAN_POINT('Ctrl Pts',(-23.534,5.29184265751413,-5.4465758210584));
#116368=CARTESIAN_POINT('Ctrl Pts',(-23.534,5.24629059068216,-5.56093558465363));
#116369=CARTESIAN_POINT('Ctrl Pts',(-23.5339999999999,5.20492644341908,
-5.67694766331998));
#116370=CARTESIAN_POINT('Ctrl Pts',(-23.5319824436158,5.20171895019276,
-8.32379158156414));
#116371=CARTESIAN_POINT('Ctrl Pts',(-23.4932005619797,5.41676778847021,
-9.12430550294336));
#116372=CARTESIAN_POINT('Ctrl Pts',(-23.4156367987076,6.2441105606237,-10.6178355852335));
#116373=CARTESIAN_POINT('Ctrl Pts',(-23.2992911537994,8.39090036149447,
-12.0161877049687));
#116374=CARTESIAN_POINT('Ctrl Pts',(-23.1829455088912,10.9421734111865,
-12.2463209198922));
#116375=CARTESIAN_POINT('Ctrl Pts',(-23.066599863983,13.3043923657925,-11.254988095828));
#116376=CARTESIAN_POINT('Ctrl Pts',(-22.9502542190748,14.9272765412854,
-9.27285603598496));
#116377=CARTESIAN_POINT('Ctrl Pts',(-22.8339085741666,15.4330667658206,
-6.76152808894962));
#116378=CARTESIAN_POINT('Ctrl Pts',(-22.7175629292584,14.7039358375933,
-4.30571513125084));
#116379=CARTESIAN_POINT('Ctrl Pts',(-22.6012172843502,12.9096844371217,
-2.47725527851035));
#116380=CARTESIAN_POINT('Ctrl Pts',(-22.484871639442,10.468080449077,-1.70188612182472));
#116381=CARTESIAN_POINT('Ctrl Pts',(-22.3685259945338,7.94764126437696,
-2.16015086439891));
#116382=CARTESIAN_POINT('Ctrl Pts',(-22.2521803496256,5.93523522075824,
-3.74534493575574));
#116383=CARTESIAN_POINT('Ctrl Pts',(-22.1358347047174,4.8994345496665,-6.08836357882409));
#116384=CARTESIAN_POINT('Ctrl Pts',(-22.0194890598092,5.08142987925019,
-8.64365526468454));
#116385=CARTESIAN_POINT('Ctrl Pts',(-21.903143414901,6.43882094024319,-10.8162231015153));
#116386=CARTESIAN_POINT('Ctrl Pts',(-21.7867977699929,8.65559788490324,
-12.1002256459208));
#116387=CARTESIAN_POINT('Ctrl Pts',(-21.6704521250846,11.2154924815527,
-12.196633040956));
#116388=CARTESIAN_POINT('Ctrl Pts',(-21.5541064801764,13.522669729074,-11.0831184026112));
#116389=CARTESIAN_POINT('Ctrl Pts',(-21.4377608352682,15.0394560589382,
-9.0187036198784));
#116390=CARTESIAN_POINT('Ctrl Pts',(-21.32141519036,15.4136427834887,-6.48460441844491));
#116391=CARTESIAN_POINT('Ctrl Pts',(-21.2050695454519,14.5560828744103,
-4.0697625184195));
#116392=CARTESIAN_POINT('Ctrl Pts',(-21.0887239005437,12.6706795512211,
-2.33877606381416));
#116393=CARTESIAN_POINT('Ctrl Pts',(-20.9723782556355,10.1876014233208,
-1.68985101778543));
#116394=CARTESIAN_POINT('Ctrl Pts',(-20.8560326107273,7.70350671639053,
-2.28420971589842));
#116395=CARTESIAN_POINT('Ctrl Pts',(-20.700905084183,5.11052115881551,-4.52263843008836));
#116396=CARTESIAN_POINT('Ctrl Pts',(-20.5069956760027,4.5360766030555,-9.14006182725829));
#116397=CARTESIAN_POINT('Ctrl Pts',(-20.2743043861863,8.77988233534782,
-12.8347906630172));
#116398=CARTESIAN_POINT('Ctrl Pts',(-20.080394978006,13.2742513752808,-11.6301196252367));
#116399=CARTESIAN_POINT('Ctrl Pts',(-19.9252674514617,15.1343798224707,
-8.75365315224294));
#116400=CARTESIAN_POINT('Ctrl Pts',(-19.8089218065535,15.3810849987625,
-6.21138539863939));
#116401=CARTESIAN_POINT('Ctrl Pts',(-19.6925761616453,14.396485337932,-3.84129168477222));
#116402=CARTESIAN_POINT('Ctrl Pts',(-19.5762305167371,12.42241195026,-2.21215263079145));
#116403=CARTESIAN_POINT('Ctrl Pts',(-19.459884871829,9.91250174166068,-1.69521825918731));
#116404=CARTESIAN_POINT('Ctrl Pts',(-19.3435392269207,7.45404862565434,
-2.41471999228771));
#116405=CARTESIAN_POINT('Ctrl Pts',(-19.2271935820125,5.61811305085138,
-4.201278060418));
#116406=CARTESIAN_POINT('Ctrl Pts',(-19.1108479371043,4.8328386716438,-6.63978700045667));
#116407=CARTESIAN_POINT('Ctrl Pts',(-18.9945022921962,5.28075752071532,
-9.1620327133916));
#116408=CARTESIAN_POINT('Ctrl Pts',(-18.878156647288,6.85772466794919,-11.1809277510202));
#116409=CARTESIAN_POINT('Ctrl Pts',(-18.7618110023798,9.1964812960346,-12.2262884221197));
#116410=CARTESIAN_POINT('Ctrl Pts',(-18.6454653574715,11.7524965873672,
-12.0547549551468));
#116411=CARTESIAN_POINT('Ctrl Pts',(-18.5291197125634,13.9306020129096,
-10.7062460945076));
#116412=CARTESIAN_POINT('Ctrl Pts',(-18.4127740676552,15.2236465040783,
-8.49476372466684));
#116413=CARTESIAN_POINT('Ctrl Pts',(-18.296428422747,15.3305499866057,-5.93523409923148));
#116414=CARTESIAN_POINT('Ctrl Pts',(-18.1800827778388,14.2264201441576,
-3.62362758976861));
#116415=CARTESIAN_POINT('Ctrl Pts',(-18.0637371329306,12.1683507297645,
-2.09819197765073));
#116416=CARTESIAN_POINT('Ctrl Pts',(-17.9473914880224,9.63554086184729,
-1.7141042706357));
#116417=CARTESIAN_POINT('Ctrl Pts',(-17.8310458431142,7.2177604705694,-2.56082133574547));
#116418=CARTESIAN_POINT('Ctrl Pts',(-17.714700198206,5.4779309504908,-4.44113880648963));
#116419=CARTESIAN_POINT('Ctrl Pts',(-17.5983545532978,4.82125271145331,
-6.91734413883624));
#116420=CARTESIAN_POINT('Ctrl Pts',(-17.4820089083896,5.40043704181473,
-9.4126399093131));
#116421=CARTESIAN_POINT('Ctrl Pts',(-17.3656593823793,7.08108558213933,
-11.3465358543532));
#116422=CARTESIAN_POINT('Ctrl Pts',(-17.2880917380051,8.67440028619388,
-11.9603779064283));
#116423=CARTESIAN_POINT('Ctrl Pts',(-17.2493059752669,9.49698545957615,
-12.0631389059803));
#116424=CARTESIAN_POINT('Ctrl Pts',(-23.6939479458674,5.47264577451099,
-8.25101021290606));
#116425=CARTESIAN_POINT('Ctrl Pts',(-23.6551660642314,5.6758713401554,-9.00751229764933));
#116426=CARTESIAN_POINT('Ctrl Pts',(-23.5776023009592,6.45772723949198,
-10.4189288773044));
#116427=CARTESIAN_POINT('Ctrl Pts',(-23.461256656051,8.48648766013054,-11.7404003289966));
#116428=CARTESIAN_POINT('Ctrl Pts',(-23.3449110111429,10.8974930521617,
-11.95788094015));
#116429=CARTESIAN_POINT('Ctrl Pts',(-23.2285653662346,13.1298384443577,
-11.0210510761709));
#116430=CARTESIAN_POINT('Ctrl Pts',(-23.1122197213265,14.6634972968383,
-9.14789560009342));
#116431=CARTESIAN_POINT('Ctrl Pts',(-22.9958740764182,15.1414794394154,
-6.77463914987075));
#116432=CARTESIAN_POINT('Ctrl Pts',(-22.8795284315101,14.4524357482022,
-4.45384550391166));
#116433=CARTESIAN_POINT('Ctrl Pts',(-22.7631827866019,12.7568313511272,
-2.72591341737859));
#116434=CARTESIAN_POINT('Ctrl Pts',(-22.6468371416937,10.4494654731035,
-1.99317365131966));
#116435=CARTESIAN_POINT('Ctrl Pts',(-22.5304914967855,8.06759871629672,
-2.42624323807267));
#116436=CARTESIAN_POINT('Ctrl Pts',(-22.4141458518773,6.16583370423474,
-3.92428416862637));
#116437=CARTESIAN_POINT('Ctrl Pts',(-22.2978002069691,5.18698081219592,
-6.13848487236893));
#116438=CARTESIAN_POINT('Ctrl Pts',(-22.1814545620609,5.35897013376373,
-8.55328795805423));
#116439=CARTESIAN_POINT('Ctrl Pts',(-22.0651089171527,6.64173254429605,
-10.6064091517207));
#116440=CARTESIAN_POINT('Ctrl Pts',(-21.9487632722445,8.73663225216978,
-11.8198179079167));
#116441=CARTESIAN_POINT('Ctrl Pts',(-21.8324176273363,11.1557851830167,
-11.9109248748051));
#116442=CARTESIAN_POINT('Ctrl Pts',(-21.7160719824281,13.3361150323902,
-10.8586306887794));
#116443=CARTESIAN_POINT('Ctrl Pts',(-21.5997263375199,14.7695092432934,
-8.90771635087327));
#116444=CARTESIAN_POINT('Ctrl Pts',(-21.4833806926117,15.1231233774711,
-6.51294059790724));
#116445=CARTESIAN_POINT('Ctrl Pts',(-21.3670350477035,14.3127116635907,
-4.23086544230325));
#116446=CARTESIAN_POINT('Ctrl Pts',(-21.2506894027953,12.5309668288262,
-2.59504771746573));
#116447=CARTESIAN_POINT('Ctrl Pts',(-21.1343437578871,10.1844070374604,
-1.98180023100471));
#116448=CARTESIAN_POINT('Ctrl Pts',(-21.0179981129789,7.83688655804795,
-2.54348139881387));
#116449=CARTESIAN_POINT('Ctrl Pts',(-20.8628705864347,5.38646198999665,
-4.6588424732551));
#116450=CARTESIAN_POINT('Ctrl Pts',(-20.6689611782544,4.84360009541132,
-9.0224023474958));
#116451=CARTESIAN_POINT('Ctrl Pts',(-20.436269888438,8.85408360854405,-12.5139969246358));
#116452=CARTESIAN_POINT('Ctrl Pts',(-20.2423604802577,13.101354589737,-11.37555807033));
#116453=CARTESIAN_POINT('Ctrl Pts',(-20.0872329537134,14.8592141479629,
-8.6572382192963));
#116454=CARTESIAN_POINT('Ctrl Pts',(-19.9708873088052,15.0923556027177,
-6.25474301688543));
#116455=CARTESIAN_POINT('Ctrl Pts',(-19.854541663897,14.16188871618,-4.01495581557319));
#116456=CARTESIAN_POINT('Ctrl Pts',(-19.7381960189888,12.2963488506932,
-2.47538597455189));
#116457=CARTESIAN_POINT('Ctrl Pts',(-19.6218503740806,9.92443219238895,
-1.986872384282));
#116458=CARTESIAN_POINT('Ctrl Pts',(-19.5055047291724,7.60114354264496,
-2.66681628847928));
#116459=CARTESIAN_POINT('Ctrl Pts',(-19.3891590842642,5.86614674533775,
-4.35515032860052));
#116460=CARTESIAN_POINT('Ctrl Pts',(-19.272813439356,5.12404634070955,-6.65959132273846));
#116461=CARTESIAN_POINT('Ctrl Pts',(-19.1564677944478,5.54733884577256,
-9.04316528580281));
#116462=CARTESIAN_POINT('Ctrl Pts',(-19.0401221495396,7.03760516418795,
-10.9510625303785));
#116463=CARTESIAN_POINT('Ctrl Pts',(-18.9237765046314,9.24777817630178,
-11.9389498186257));
#116464=CARTESIAN_POINT('Ctrl Pts',(-18.8074308597232,11.6632650840089,
-11.776847171935));
#116465=CARTESIAN_POINT('Ctrl Pts',(-18.6910852148151,13.7216194126565,
-10.5024786230275));
#116466=CARTESIAN_POINT('Ctrl Pts',(-18.5747395699068,14.9435729941127,
-8.4125823970192));
#116467=CARTESIAN_POINT('Ctrl Pts',(-18.4583939249987,15.0445989790936,
-5.99377437145986));
#116468=CARTESIAN_POINT('Ctrl Pts',(-18.3420482800905,14.0011736177956,
-3.80925877864935));
#116469=CARTESIAN_POINT('Ctrl Pts',(-18.2257026351823,12.0562557831971,
-2.36769081850622));
#116470=CARTESIAN_POINT('Ctrl Pts',(-18.1093569902741,9.66269847686509,
-2.00472005270053));
#116471=CARTESIAN_POINT('Ctrl Pts',(-17.9930113453659,7.37784638672052,
-2.80488505650165));
#116472=CARTESIAN_POINT('Ctrl Pts',(-17.8766657004577,5.73367178352352,
-4.58182365632809));
#116473=CARTESIAN_POINT('Ctrl Pts',(-17.7603200555495,5.11309737054954,
-6.92188851484443));
#116474=CARTESIAN_POINT('Ctrl Pts',(-17.6439744106413,5.66043844940817,
-9.27999422918914));
#116475=CARTESIAN_POINT('Ctrl Pts',(-17.527624884631,7.24868581215954,-11.1075655868224));
#116476=CARTESIAN_POINT('Ctrl Pts',(-17.4500572402568,8.75440090727327,
-11.687658923985));
#116477=CARTESIAN_POINT('Ctrl Pts',(-17.4112714775186,9.53176077813031,
-11.7847701775375));
#116478=CARTESIAN_POINT('Ctrl Pts',(-23.8559134481191,5.74357259882922,
-8.17822884424796));
#116479=CARTESIAN_POINT('Ctrl Pts',(-23.817131566483,5.93497489184058,-8.8907190923553));
#116480=CARTESIAN_POINT('Ctrl Pts',(-23.7395678032109,6.67134391836025,
-10.2200221693753));
#116481=CARTESIAN_POINT('Ctrl Pts',(-23.6232221583027,8.58207495876662,
-11.4646129530245));
#116482=CARTESIAN_POINT('Ctrl Pts',(-23.5068765133945,10.852812693137,-11.6694409604076));
#116483=CARTESIAN_POINT('Ctrl Pts',(-23.3905308684863,12.9552845229227,
-10.7871140565138));
#116484=CARTESIAN_POINT('Ctrl Pts',(-23.2741852235781,14.3997180523911,
-9.0229351642019));
#116485=CARTESIAN_POINT('Ctrl Pts',(-23.1578395786699,14.8498921130101,
-6.78775021079188));
#116486=CARTESIAN_POINT('Ctrl Pts',(-23.0414939337617,14.2009356588109,
-4.60197587657248));
#116487=CARTESIAN_POINT('Ctrl Pts',(-22.9251482888536,12.6039782651327,
-2.97457155624683));
#116488=CARTESIAN_POINT('Ctrl Pts',(-22.8088026439453,10.43085049713,-2.28446118081461));
#116489=CARTESIAN_POINT('Ctrl Pts',(-22.6924569990372,8.18755616821649,
-2.69233561174642));
#116490=CARTESIAN_POINT('Ctrl Pts',(-22.576111354129,6.39643218771124,-4.10322340149701));
#116491=CARTESIAN_POINT('Ctrl Pts',(-22.4597657092208,5.47452707472534,
-6.18860616591375));
#116492=CARTESIAN_POINT('Ctrl Pts',(-22.3434200643126,5.63651038827726,
-8.46292065142394));
#116493=CARTESIAN_POINT('Ctrl Pts',(-22.2270744194044,6.84464414834892,
-10.3965952019259));
#116494=CARTESIAN_POINT('Ctrl Pts',(-22.1107287744962,8.81766661943629,
-11.5394101699127));
#116495=CARTESIAN_POINT('Ctrl Pts',(-21.994383129588,11.0960778844808,-11.6252167086543));
#116496=CARTESIAN_POINT('Ctrl Pts',(-21.8780374846798,13.1495603357064,
-10.6341429749476));
#116497=CARTESIAN_POINT('Ctrl Pts',(-21.7616918397716,14.4995624276486,
-8.79672908186814));
#116498=CARTESIAN_POINT('Ctrl Pts',(-21.6453461948634,14.8326039714535,
-6.54127677736955));
#116499=CARTESIAN_POINT('Ctrl Pts',(-21.5290005499552,14.0693404527711,
-4.39196836618699));
#116500=CARTESIAN_POINT('Ctrl Pts',(-21.412654905047,12.3912541064312,-2.85131937111729));
#116501=CARTESIAN_POINT('Ctrl Pts',(-21.2963092601388,10.1812126516,-2.27374944422398));
#116502=CARTESIAN_POINT('Ctrl Pts',(-21.1799636152306,7.97026639970535,
-2.80275308172933));
#116503=CARTESIAN_POINT('Ctrl Pts',(-21.0248360886864,5.66240282117781,
-4.79504651642184));
#116504=CARTESIAN_POINT('Ctrl Pts',(-20.830926680506,5.15112358776711,-8.90474286773331));
#116505=CARTESIAN_POINT('Ctrl Pts',(-20.5982353906897,8.9282848817403,-12.1932031862544));
#116506=CARTESIAN_POINT('Ctrl Pts',(-20.4043259825093,12.9284578041932,
-11.1209965154232));
#116507=CARTESIAN_POINT('Ctrl Pts',(-20.2491984559651,14.5840484734553,
-8.56082328634967));
#116508=CARTESIAN_POINT('Ctrl Pts',(-20.1328528110569,14.8036262066728,
-6.29810063513147));
#116509=CARTESIAN_POINT('Ctrl Pts',(-20.0165071661487,13.927292094428,-4.18861994637416));
#116510=CARTESIAN_POINT('Ctrl Pts',(-19.9001615212405,12.1702857511264,
-2.73861931831233));
#116511=CARTESIAN_POINT('Ctrl Pts',(-19.7838158763323,9.93636264311722,
-2.2785265093767));
#116512=CARTESIAN_POINT('Ctrl Pts',(-19.6674702314241,7.74823845963558,
-2.91891258467084));
#116513=CARTESIAN_POINT('Ctrl Pts',(-19.5511245865159,6.1141804398241,-4.50902259678305));
#116514=CARTESIAN_POINT('Ctrl Pts',(-19.4347789416077,5.41525400977531,
-6.67939564502024));
#116515=CARTESIAN_POINT('Ctrl Pts',(-19.3184332966995,5.81392017082977,
-8.92429785821404));
#116516=CARTESIAN_POINT('Ctrl Pts',(-19.2020876517913,7.21748566042671,
-10.7211973097368));
#116517=CARTESIAN_POINT('Ctrl Pts',(-19.0857420068831,9.29907505656898,
-11.6516112151316));
#116518=CARTESIAN_POINT('Ctrl Pts',(-18.9693963619749,11.5740335806506,
-11.4989393887233));
#116519=CARTESIAN_POINT('Ctrl Pts',(-18.8530507170667,13.5126368124033,
-10.2987111515474));
#116520=CARTESIAN_POINT('Ctrl Pts',(-18.7367050721585,14.663499484147,-8.33040106937155));
#116521=CARTESIAN_POINT('Ctrl Pts',(-18.6203594272503,14.7586479715815,
-6.05231464368824));
#116522=CARTESIAN_POINT('Ctrl Pts',(-18.5040137823422,13.7759270914335,
-3.99488996753009));
#116523=CARTESIAN_POINT('Ctrl Pts',(-18.3876681374339,11.9441608366297,
-2.63718965936172));
#116524=CARTESIAN_POINT('Ctrl Pts',(-18.2713224925258,9.6898560918829,-2.29533583476536));
#116525=CARTESIAN_POINT('Ctrl Pts',(-18.1549768476175,7.53793230287164,
-3.04894877725783));
#116526=CARTESIAN_POINT('Ctrl Pts',(-18.0386312027094,5.98941261655623,
-4.72250850616656));
#116527=CARTESIAN_POINT('Ctrl Pts',(-17.9222855578012,5.40494202964576,
-6.92643289085262));
#116528=CARTESIAN_POINT('Ctrl Pts',(-17.805939912893,5.9204398570016,-9.14734854906519));
#116529=CARTESIAN_POINT('Ctrl Pts',(-17.6895903868827,7.41628604217975,
-10.8685953192918));
#116530=CARTESIAN_POINT('Ctrl Pts',(-17.6120227425084,8.83440152835267,
-11.4149399415416));
#116531=CARTESIAN_POINT('Ctrl Pts',(-17.5732369797703,9.56653609668444,
-11.5064014490947));
#116532=CARTESIAN_POINT('Ctrl Pts',(-24.0178789503708,6.01449942314746,
-8.10544747558987));
#116533=CARTESIAN_POINT('Ctrl Pts',(-23.9790970687347,6.19407844352577,
-8.77392588706126));
#116534=CARTESIAN_POINT('Ctrl Pts',(-23.9015333054626,6.88496059722852,
-10.021115461446));
#116535=CARTESIAN_POINT('Ctrl Pts',(-23.7851876605544,8.6776622574027,-11.1888255770524));
#116536=CARTESIAN_POINT('Ctrl Pts',(-23.6688420156462,10.8081323341124,
-11.3810009806654));
#116537=CARTESIAN_POINT('Ctrl Pts',(-23.552496370738,12.7807306014878,-10.5531770368568));
#116538=CARTESIAN_POINT('Ctrl Pts',(-23.4361507258298,14.135938807944,-8.89797472831037));
#116539=CARTESIAN_POINT('Ctrl Pts',(-23.3198050809216,14.558304786605,-6.800861271713));
#116540=CARTESIAN_POINT('Ctrl Pts',(-23.2034594360134,13.9494355694199,
-4.7501062492333));
#116541=CARTESIAN_POINT('Ctrl Pts',(-23.0871137911052,12.4511251791381,
-3.22322969511507));
#116542=CARTESIAN_POINT('Ctrl Pts',(-22.970768146197,10.4122355211566,-2.57574871030957));
#116543=CARTESIAN_POINT('Ctrl Pts',(-22.8544225012888,8.30751362013623,
-2.95842798542018));
#116544=CARTESIAN_POINT('Ctrl Pts',(-22.7380768563806,6.62703067118774,
-4.28216263436764));
#116545=CARTESIAN_POINT('Ctrl Pts',(-22.6217312114725,5.76207333725475,
-6.23872745945858));
#116546=CARTESIAN_POINT('Ctrl Pts',(-22.5053855665642,5.91405064279082,
-8.37255334479363));
#116547=CARTESIAN_POINT('Ctrl Pts',(-22.3890399216561,7.04755575240179,
-10.1867812521313));
#116548=CARTESIAN_POINT('Ctrl Pts',(-22.2726942767479,8.89870098670282,
-11.2590024319086));
#116549=CARTESIAN_POINT('Ctrl Pts',(-22.1563486318397,11.0363705859449,
-11.3395085425033));
#116550=CARTESIAN_POINT('Ctrl Pts',(-22.0400029869315,12.9630056390227,
-10.4096552611159));
#116551=CARTESIAN_POINT('Ctrl Pts',(-21.9236573420233,14.2296156120038,
-8.68574181286299));
#116552=CARTESIAN_POINT('Ctrl Pts',(-21.8073116971151,14.5420845654359,
-6.56961295683188));
#116553=CARTESIAN_POINT('Ctrl Pts',(-21.6909660522069,13.8259692419515,
-4.55307129007074));
#116554=CARTESIAN_POINT('Ctrl Pts',(-21.5746204072987,12.2515413840362,
-3.10759102476887));
#116555=CARTESIAN_POINT('Ctrl Pts',(-21.4582747623905,10.1780182657396,
-2.56569865744326));
#116556=CARTESIAN_POINT('Ctrl Pts',(-21.3419291174823,8.10364624136277,
-3.06202476464478));
#116557=CARTESIAN_POINT('Ctrl Pts',(-21.186801590938,5.93834365235895,-4.93125055958858));
#116558=CARTESIAN_POINT('Ctrl Pts',(-20.9928921827577,5.45864708012292,
-8.78708338797083));
#116559=CARTESIAN_POINT('Ctrl Pts',(-20.7602008929413,9.00248615493654,
-11.8724094478728));
#116560=CARTESIAN_POINT('Ctrl Pts',(-20.566291484761,12.7555610186494,-10.8664349605165));
#116561=CARTESIAN_POINT('Ctrl Pts',(-20.4111639582168,14.3088827989476,
-8.46440835340305));
#116562=CARTESIAN_POINT('Ctrl Pts',(-20.2948183133085,14.514896810628,-6.34145825337751));
#116563=CARTESIAN_POINT('Ctrl Pts',(-20.1784726684004,13.6926954726759,
-4.36228407717513));
#116564=CARTESIAN_POINT('Ctrl Pts',(-20.0621270234921,12.0442226515596,
-3.00185266207277));
#116565=CARTESIAN_POINT('Ctrl Pts',(-19.945781378584,9.94829309384551,-2.57018063447138));
#116566=CARTESIAN_POINT('Ctrl Pts',(-19.8294357336758,7.89533337662619,
-3.17100888086241));
#116567=CARTESIAN_POINT('Ctrl Pts',(-19.7130900887676,6.36221413431046,
-4.66289486496558));
#116568=CARTESIAN_POINT('Ctrl Pts',(-19.5967444438594,5.70646167884105,
-6.69919996730202));
#116569=CARTESIAN_POINT('Ctrl Pts',(-19.4803987989512,6.08050149588701,
-8.80543043062526));
#116570=CARTESIAN_POINT('Ctrl Pts',(-19.364053154043,7.39736615666546,-10.4913320890951));
#116571=CARTESIAN_POINT('Ctrl Pts',(-19.2477075091348,9.35037193683615,
-11.3642726116376));
#116572=CARTESIAN_POINT('Ctrl Pts',(-19.1313618642266,11.4848020772924,
-11.2210316055115));
#116573=CARTESIAN_POINT('Ctrl Pts',(-19.0150162193184,13.30365421215,-10.0949436800673));
#116574=CARTESIAN_POINT('Ctrl Pts',(-18.8986705744102,14.3834259741814,
-8.2482197417239));
#116575=CARTESIAN_POINT('Ctrl Pts',(-18.782324929502,14.4726969640693,-6.1108549159166));
#116576=CARTESIAN_POINT('Ctrl Pts',(-18.6659792845938,13.5506805650714,
-4.18052115641083));
#116577=CARTESIAN_POINT('Ctrl Pts',(-18.5496336396856,11.8320658900623,
-2.90668850021721));
#116578=CARTESIAN_POINT('Ctrl Pts',(-18.4332879947774,9.7170137069007,-2.58595161683019));
#116579=CARTESIAN_POINT('Ctrl Pts',(-18.3169423498692,7.69801821902275,
-3.293012498014));
#116580=CARTESIAN_POINT('Ctrl Pts',(-18.200596704961,6.24515344958894,-4.86319335600501));
#116581=CARTESIAN_POINT('Ctrl Pts',(-18.0842510600528,5.69678668874198,
-6.93097726686083));
#116582=CARTESIAN_POINT('Ctrl Pts',(-17.9679054151447,6.18044126459504,
-9.01470286894122));
#116583=CARTESIAN_POINT('Ctrl Pts',(-17.8515558891343,7.58388627219995,
-10.6296250517611));
#116584=CARTESIAN_POINT('Ctrl Pts',(-17.7739882447601,8.91440214943207,
-11.1422209590983));
#116585=CARTESIAN_POINT('Ctrl Pts',(-17.735202482022,9.6013114152386,-11.2280327206518));
#116586=CARTESIAN_POINT('Ctrl Pts',(-17.734,9.60084442449481,-11.2300936493755));
#116587=CARTESIAN_POINT('Ctrl Pts',(-17.734,9.47184184893834,-11.2265276083404));
#116588=CARTESIAN_POINT('Ctrl Pts',(-17.734,9.34319367231545,-11.2169788959015));
#116589=CARTESIAN_POINT('Ctrl Pts',(-17.734,9.21527281511486,-11.2016549822556));
#116590=CARTESIAN_POINT('Ctrl Pts',(-17.734,9.08501147085063,-11.1860506966482));
#116591=CARTESIAN_POINT('Ctrl Pts',(-17.734,8.95550358630314,-11.1644579949374));
#116592=CARTESIAN_POINT('Ctrl Pts',(-17.734,8.82713205817655,-11.1370431678773));
#116593=CARTESIAN_POINT('Ctrl Pts',(-17.734,8.77054626721239,-11.1249587929697));
#116594=CARTESIAN_POINT('Ctrl Pts',(-17.734,8.7141811982412,-11.1117424824817));
#116595=CARTESIAN_POINT('Ctrl Pts',(-17.7339999999999,8.65806956321802,
-11.0974052780753));
#116596=CARTESIAN_POINT('Ctrl Pts',(-17.7339999999999,8.63585998151805,
-11.0917304601435));
#116597=CARTESIAN_POINT('Ctrl Pts',(-17.734,8.61369010565667,-11.0858800148832));
#116598=CARTESIAN_POINT('Ctrl Pts',(-17.734,8.59156197215374,-11.0798545436473));
#116599=CARTESIAN_POINT('Ctrl Pts',(-17.734,8.56803675576561,-11.073448647974));
#116600=CARTESIAN_POINT('Ctrl Pts',(-17.734,8.54456657927922,-11.0668470333961));
#116601=CARTESIAN_POINT('Ctrl Pts',(-17.734,8.52115967302967,-11.0600525704303));
#116602=CARTESIAN_POINT('Ctrl Pts',(-17.734,8.39238352917026,-11.0226719473357));
#116603=CARTESIAN_POINT('Ctrl Pts',(-17.7339999999999,8.26546690752475,
-10.9794433217256));
#116604=CARTESIAN_POINT('Ctrl Pts',(-17.7339999999999,8.14080691439625,
-10.9305498903925));
#116605=CARTESIAN_POINT('Ctrl Pts',(-17.7339999999999,8.04196929345981,
-10.8917843625668));
#116606=CARTESIAN_POINT('Ctrl Pts',(-17.734,7.94454991934812,-10.8494567334459));
#116607=CARTESIAN_POINT('Ctrl Pts',(-17.7339999999999,7.84874780521352,
-10.8036350740797));
#116608=CARTESIAN_POINT('Ctrl Pts',(-17.7339999999999,7.8007073644388,-10.780657577885));
#116609=CARTESIAN_POINT('Ctrl Pts',(-17.734,7.75307363883164,-10.7568011656462));
#116610=CARTESIAN_POINT('Ctrl Pts',(-17.734,7.70587215411362,-10.7320725309682));
#116611=CARTESIAN_POINT('Ctrl Pts',(-17.734,7.6793174922842,-10.7181606691847));
#116612=CARTESIAN_POINT('Ctrl Pts',(-17.734,7.65289964014865,-10.7039727286759));
#116613=CARTESIAN_POINT('Ctrl Pts',(-17.734,7.6266232029969,-10.6895097288812));
#116614=CARTESIAN_POINT('Ctrl Pts',(-17.734,7.60953423118557,-10.6801036669266));
#116615=CARTESIAN_POINT('Ctrl Pts',(-17.734,7.59250626485928,-10.6705818595696));
#116616=CARTESIAN_POINT('Ctrl Pts',(-17.734,7.57555065957241,-10.660950526036));
#116617=CARTESIAN_POINT('Ctrl Pts',(-17.734,7.57223521227194,-10.6590672444767));
#116618=CARTESIAN_POINT('Ctrl Pts',(-17.734,7.56892242572952,-10.6571797172604));
#116619=CARTESIAN_POINT('Ctrl Pts',(-17.734,7.56561230852364,-10.655287949029));
#116620=CARTESIAN_POINT('Ctrl Pts',(-17.734,7.44527804479261,-10.5865155995581));
#116621=CARTESIAN_POINT('Ctrl Pts',(-17.734,7.32847088871136,-10.5121436774441));
#116622=CARTESIAN_POINT('Ctrl Pts',(-17.734,7.21544353549546,-10.4326038138175));
#116623=CARTESIAN_POINT('Ctrl Pts',(-17.734,7.10471415648964,-10.3546810857788));
#116624=CARTESIAN_POINT('Ctrl Pts',(-17.734,6.99761187192383,-10.2717977527096));
#116625=CARTESIAN_POINT('Ctrl Pts',(-17.734,6.89438670712412,-10.1843052779668));
#116626=CARTESIAN_POINT('Ctrl Pts',(-17.734,6.78794818419843,-10.0940891974518));
#116627=CARTESIAN_POINT('Ctrl Pts',(-17.734,6.68563112333944,-9.9989722894686));
#116628=CARTESIAN_POINT('Ctrl Pts',(-17.734,6.58773359226506,-9.89928785076242));
#116629=CARTESIAN_POINT('Ctrl Pts',(-17.734,6.48983606119067,-9.79960341205624));
#116630=CARTESIAN_POINT('Ctrl Pts',(-17.734,6.39635732386312,-9.69535089177204));
#116631=CARTESIAN_POINT('Ctrl Pts',(-17.734,6.3076305292093,-9.58681889811916));
#116632=CARTESIAN_POINT('Ctrl Pts',(-17.734,6.29613696047738,-9.57275978628572));
#116633=CARTESIAN_POINT('Ctrl Pts',(-17.734,6.2847217875374,-9.55862705010366));
#116634=CARTESIAN_POINT('Ctrl Pts',(-17.734,6.27339033844863,-9.54442698291117));
#116635=CARTESIAN_POINT('Ctrl Pts',(-17.734,6.18608899588886,-9.43502482960916));
#116636=CARTESIAN_POINT('Ctrl Pts',(-17.734,6.10395851094937,-9.32188720168948));
#116637=CARTESIAN_POINT('Ctrl Pts',(-17.734,6.02725312841167,-9.20538411899327));
#116638=CARTESIAN_POINT('Ctrl Pts',(-17.734,6.00879365458167,-9.17734716076432));
#116639=CARTESIAN_POINT('Ctrl Pts',(-17.734,5.99064847657934,-9.14911508036603));
#116640=CARTESIAN_POINT('Ctrl Pts',(-17.734,5.97282135213961,-9.12069264219457));
#116641=CARTESIAN_POINT('Ctrl Pts',(-17.734,5.8993219360575,-9.00350982809044));
#116642=CARTESIAN_POINT('Ctrl Pts',(-17.734,5.8312260111049,-8.88309435288586));
#116643=CARTESIAN_POINT('Ctrl Pts',(-17.734,5.76858202624986,-8.7598729906184));
#116644=CARTESIAN_POINT('Ctrl Pts',(-17.734,5.7037197407521,-8.63228820817986));
#116645=CARTESIAN_POINT('Ctrl Pts',(-17.734,5.64470175837656,-8.50169476853212));
#116646=CARTESIAN_POINT('Ctrl Pts',(-17.734,5.59162577020733,-8.36852853807731));
#116647=CARTESIAN_POINT('Ctrl Pts',(-17.734,5.5385497820381,-8.23536230762251));
#116648=CARTESIAN_POINT('Ctrl Pts',(-17.734,5.49141540954946,-8.09962248344302));
#116649=CARTESIAN_POINT('Ctrl Pts',(-17.734,5.45037050417322,-7.96171819969766));
#116650=CARTESIAN_POINT('Ctrl Pts',(-17.734,5.44370883975598,-7.93933607817511));
#116651=CARTESIAN_POINT('Ctrl Pts',(-17.734,5.43720810243115,-7.91689789280803));
#116652=CARTESIAN_POINT('Ctrl Pts',(-17.734,5.43087453779524,-7.89442610997133));
#116653=CARTESIAN_POINT('Ctrl Pts',(-17.734,5.39210005996093,-7.75685245349387));
#116654=CARTESIAN_POINT('Ctrl Pts',(-17.734,5.35952760976202,-7.61782263146663));
#116655=CARTESIAN_POINT('Ctrl Pts',(-17.734,5.33320157525561,-7.47778296854049));
#116656=CARTESIAN_POINT('Ctrl Pts',(-17.734,5.30659247764124,-7.33623756944981));
#116657=CARTESIAN_POINT('Ctrl Pts',(-17.734,5.28636445801933,-7.19365980485496));
#116658=CARTESIAN_POINT('Ctrl Pts',(-17.734,5.27260711226718,-7.05048093600343));
#116659=CARTESIAN_POINT('Ctrl Pts',(-17.734,5.26856672905835,-7.00843085541456));
#116660=CARTESIAN_POINT('Ctrl Pts',(-17.734,5.26508476885711,-6.96632877289766));
#116661=CARTESIAN_POINT('Ctrl Pts',(-17.734,5.26216428318299,-6.92418527139126));
#116662=CARTESIAN_POINT('Ctrl Pts',(-17.734,5.25225669184947,-6.78121569821777));
#116663=CARTESIAN_POINT('Ctrl Pts',(-17.734,5.24880693790302,-6.6377701872535));
#116664=CARTESIAN_POINT('Ctrl Pts',(-17.734,5.25169843615224,-6.49425035729587));
#116665=CARTESIAN_POINT('Ctrl Pts',(-17.734,5.25418827323925,-6.37066702279183));
#116666=CARTESIAN_POINT('Ctrl Pts',(-17.734,5.26138083595832,-6.24702806280391));
#116667=CARTESIAN_POINT('Ctrl Pts',(-17.734,5.27323254549849,-6.123587571864));
#116668=CARTESIAN_POINT('Ctrl Pts',(-17.734,5.27508188116906,-6.10432597063131));
#116669=CARTESIAN_POINT('Ctrl Pts',(-17.734,5.27704501035193,-6.08506650230671));
#116670=CARTESIAN_POINT('Ctrl Pts',(-17.734,5.27912085414996,-6.06581909013264));
#116671=CARTESIAN_POINT('Ctrl Pts',(-17.734,5.29479715330724,-5.9204670209976));
#116672=CARTESIAN_POINT('Ctrl Pts',(-17.734,5.31686509682758,-5.77608379440673));
#116673=CARTESIAN_POINT('Ctrl Pts',(-17.734,5.3451374958677,-5.63308999580944));
#116674=CARTESIAN_POINT('Ctrl Pts',(-17.734,5.37370011527558,-5.48862834466948));
#116675=CARTESIAN_POINT('Ctrl Pts',(-17.734,5.40859521043849,-5.3455840407847));
#116676=CARTESIAN_POINT('Ctrl Pts',(-17.734,5.44968220916162,-5.20437948138385));
#116677=CARTESIAN_POINT('Ctrl Pts',(-17.734,5.49084209471425,-5.06292443027113));
#116678=CARTESIAN_POINT('Ctrl Pts',(-17.734,5.53821592683283,-4.92331485930307));
#116679=CARTESIAN_POINT('Ctrl Pts',(-17.734,5.59171431219504,-4.78597586954203));
#116680=CARTESIAN_POINT('Ctrl Pts',(-17.734,5.62179155281002,-4.70876273847473));
#116681=CARTESIAN_POINT('Ctrl Pts',(-17.734,5.65380556167174,-4.63226736332771));
#116682=CARTESIAN_POINT('Ctrl Pts',(-17.734,5.68774754568469,-4.55656680513933));
#116683=CARTESIAN_POINT('Ctrl Pts',(-17.734,5.73801817128877,-4.44444859728045));
#116684=CARTESIAN_POINT('Ctrl Pts',(-17.734,5.7925169840286,-4.3340732964859));
#116685=CARTESIAN_POINT('Ctrl Pts',(-17.734,5.85109760638757,-4.22562345682715));
#116686=CARTESIAN_POINT('Ctrl Pts',(-23.534,5.20509380555676,-8.32288496556915));
#116687=CARTESIAN_POINT('Ctrl Pts',(-23.534,5.25448034822734,-8.46102114255292));
#116688=CARTESIAN_POINT('Ctrl Pts',(-23.534,5.30984160896072,-8.59666377487394));
#116689=CARTESIAN_POINT('Ctrl Pts',(-23.534,5.37090550416415,-8.72949042856159));
#116690=CARTESIAN_POINT('Ctrl Pts',(-23.534,5.43261983427461,-8.86373191325298));
#116691=CARTESIAN_POINT('Ctrl Pts',(-23.534,5.50015936697304,-8.99509777454744));
#116692=CARTESIAN_POINT('Ctrl Pts',(-23.534,5.57328932777698,-9.12322955613377));
#116693=CARTESIAN_POINT('Ctrl Pts',(-23.534,5.64611803491243,-9.25083350796567));
#116694=CARTESIAN_POINT('Ctrl Pts',(-23.534,5.72449172920252,-9.3752305570872));
#116695=CARTESIAN_POINT('Ctrl Pts',(-23.534,5.80821663861272,-9.49603209735779));
#116696=CARTESIAN_POINT('Ctrl Pts',(-23.534,5.89053472310169,-9.61480381617415));
#116697=CARTESIAN_POINT('Ctrl Pts',(-23.534,5.9780262364579,-9.73010029320117));
#116698=CARTESIAN_POINT('Ctrl Pts',(-23.534,6.07053600540052,-9.84151116210382));
#116699=CARTESIAN_POINT('Ctrl Pts',(-23.534,6.09530240287576,-9.87133769711567));
#116700=CARTESIAN_POINT('Ctrl Pts',(-23.534,6.12042860826526,-9.90088549058186));
#116701=CARTESIAN_POINT('Ctrl Pts',(-23.534,6.14591193093455,-9.93014609427624));
#116702=CARTESIAN_POINT('Ctrl Pts',(-23.534,6.15955451065975,-9.94581085369119));
#116703=CARTESIAN_POINT('Ctrl Pts',(-23.534,6.1732994431912,-9.9613932992639));
#116704=CARTESIAN_POINT('Ctrl Pts',(-23.534,6.18714632818517,-9.97689210391278));
#116705=CARTESIAN_POINT('Ctrl Pts',(-23.534,6.19947043338816,-9.99068646265098));
#116706=CARTESIAN_POINT('Ctrl Pts',(-23.534,6.21187374698249,-10.0044127646295));
#116707=CARTESIAN_POINT('Ctrl Pts',(-23.534,6.2243484693293,-10.0180621311511));
#116708=CARTESIAN_POINT('Ctrl Pts',(-23.534,6.32643586438779,-10.1297622743404));
#116709=CARTESIAN_POINT('Ctrl Pts',(-23.534,6.43344023196213,-10.2364692341204));
#116710=CARTESIAN_POINT('Ctrl Pts',(-23.534,6.54511720413425,-10.3377902027729));
#116711=CARTESIAN_POINT('Ctrl Pts',(-23.534,6.65173379038044,-10.4345200440534));
#116712=CARTESIAN_POINT('Ctrl Pts',(-23.534,6.76261007331512,-10.5263410649745));
#116713=CARTESIAN_POINT('Ctrl Pts',(-23.534,6.87736332873695,-10.6130492088598));
#116714=CARTESIAN_POINT('Ctrl Pts',(-23.534,6.99147784436095,-10.6992747177028));
#116715=CARTESIAN_POINT('Ctrl Pts',(-23.534,7.10942705472827,-10.7804443794051));
#116716=CARTESIAN_POINT('Ctrl Pts',(-23.534,7.23085436780316,-10.8563105129995));
#116717=CARTESIAN_POINT('Ctrl Pts',(-23.534,7.33613170341564,-10.9220863603421));
#116718=CARTESIAN_POINT('Ctrl Pts',(-23.534,7.44402406928361,-10.9838750073585));
#116719=CARTESIAN_POINT('Ctrl Pts',(-23.534,7.55430465571588,-11.0414837770386));
#116720=CARTESIAN_POINT('Ctrl Pts',(-23.534,7.58853359014114,-11.059364411006));
#116721=CARTESIAN_POINT('Ctrl Pts',(-23.534,7.62299261107083,-11.0768421517888));
#116722=CARTESIAN_POINT('Ctrl Pts',(-23.534,7.65767495108206,-11.0939106313755));
#116723=CARTESIAN_POINT('Ctrl Pts',(-23.534,7.68146530654451,-11.1056187570799));
#116724=CARTESIAN_POINT('Ctrl Pts',(-23.534,7.70536587584369,-11.1171366355578));
#116725=CARTESIAN_POINT('Ctrl Pts',(-23.534,7.72934494066839,-11.1284484864467));
#116726=CARTESIAN_POINT('Ctrl Pts',(-23.534,7.85661864731227,-11.1884884088606));
#116727=CARTESIAN_POINT('Ctrl Pts',(-23.5339999999999,7.9862331583221,-11.2427954978079));
#116728=CARTESIAN_POINT('Ctrl Pts',(-23.534,8.11783022540238,-11.2911803845139));
#116729=CARTESIAN_POINT('Ctrl Pts',(-23.534,8.24839999272988,-11.3391875592901));
#116730=CARTESIAN_POINT('Ctrl Pts',(-23.534,8.3809222148787,-11.381364838059));
#116731=CARTESIAN_POINT('Ctrl Pts',(-23.534,8.51505911926546,-11.4174776459003));
#116732=CARTESIAN_POINT('Ctrl Pts',(-23.534,8.54046938034511,-11.4243186855065));
#116733=CARTESIAN_POINT('Ctrl Pts',(-23.534,8.56593760260245,-11.430941947981));
#116734=CARTESIAN_POINT('Ctrl Pts',(-23.534,8.59146150656055,-11.4373456266197));
#116735=CARTESIAN_POINT('Ctrl Pts',(-23.534,8.72699587126349,-11.4713497710281));
#116736=CARTESIAN_POINT('Ctrl Pts',(-23.534,8.86410085374639,-11.4991663722465));
#116737=CARTESIAN_POINT('Ctrl Pts',(-23.534,9.00234645392461,-11.5207487445334));
#116738=CARTESIAN_POINT('Ctrl Pts',(-23.534,9.11948261257154,-11.5390355918611));
#116739=CARTESIAN_POINT('Ctrl Pts',(-23.534,9.23743788363359,-11.5528458391875));
#116740=CARTESIAN_POINT('Ctrl Pts',(-23.534,9.35594315836301,-11.5621227489502));
#116741=CARTESIAN_POINT('Ctrl Pts',(-23.534,9.3862114590886,-11.5644922324617));
#116742=CARTESIAN_POINT('Ctrl Pts',(-23.534,9.41651558906433,-11.5665658392786));
#116743=CARTESIAN_POINT('Ctrl Pts',(-23.534,9.44685094557672,-11.5683423557483));
#116744=CARTESIAN_POINT('Ctrl Pts',(-23.534,9.46479541432074,-11.5693932299733));
#116745=CARTESIAN_POINT('Ctrl Pts',(-23.534,9.48274095025219,-11.5703395658612));
#116746=CARTESIAN_POINT('Ctrl Pts',(-23.534,9.50068594451741,-11.5711814160656));
#116747=CARTESIAN_POINT('Ctrl Pts',(-23.534,9.6376789645452,-11.5776081443338));
#116748=CARTESIAN_POINT('Ctrl Pts',(-23.534,9.77465402965029,-11.5779506548684));
#116749=CARTESIAN_POINT('Ctrl Pts',(-23.534,9.91120575942691,-11.572220826072));
#116750=CARTESIAN_POINT('Ctrl Pts',(-23.534,10.0465379651975,-11.5665421695586));
#116751=CARTESIAN_POINT('Ctrl Pts',(-23.534,10.1814551280808,-11.5548989762821));
#116752=CARTESIAN_POINT('Ctrl Pts',(-23.534,10.315554055898,-11.5372529906654));
#116753=CARTESIAN_POINT('Ctrl Pts',(-23.534,10.4488851811598,-11.5197080396584));
#116754=CARTESIAN_POINT('Ctrl Pts',(-23.534,10.5814081302488,-11.4962287057312));
#116755=CARTESIAN_POINT('Ctrl Pts',(-23.534,10.7127070778146,-11.466730168397));
#116756=CARTESIAN_POINT('Ctrl Pts',(-23.5339999999999,10.7477535156779,
-11.4588563912274));
#116757=CARTESIAN_POINT('Ctrl Pts',(-23.534,10.7827126062386,-11.4505535095437));
#116758=CARTESIAN_POINT('Ctrl Pts',(-23.534,10.8175761048042,-11.4418193551064));
#116759=CARTESIAN_POINT('Ctrl Pts',(-23.534,10.9043442667858,-11.4200818199142));
#116760=CARTESIAN_POINT('Ctrl Pts',(-23.534,10.9905208003715,-11.3956733994087));
#116761=CARTESIAN_POINT('Ctrl Pts',(-23.534,11.0759855672366,-11.3686310737129));
#116762=CARTESIAN_POINT('Ctrl Pts',(-23.534,11.1080452454195,-11.3584869138336));
#116763=CARTESIAN_POINT('Ctrl Pts',(-23.534,11.1400046970052,-11.3479720510328));
#116764=CARTESIAN_POINT('Ctrl Pts',(-23.534,11.1718573159444,-11.3370881949364));
#116765=CARTESIAN_POINT('Ctrl Pts',(-23.534,11.1899003611931,-11.3309229904864));
#116766=CARTESIAN_POINT('Ctrl Pts',(-23.534,11.2079056979589,-11.3246405183814));
#116767=CARTESIAN_POINT('Ctrl Pts',(-23.534,11.2258644852499,-11.3182440453307));
#116768=CARTESIAN_POINT('Ctrl Pts',(-23.534,11.3524381725535,-11.2731616482488));
#116769=CARTESIAN_POINT('Ctrl Pts',(-23.534,11.4768170268761,-11.2223807678744));
#116770=CARTESIAN_POINT('Ctrl Pts',(-23.534,11.5986229667083,-11.1660898819115));
#116771=CARTESIAN_POINT('Ctrl Pts',(-23.534,11.7193673208413,-11.1102895927094));
#116772=CARTESIAN_POINT('Ctrl Pts',(-23.534,11.8375840316722,-11.0490744065899));
#116773=CARTESIAN_POINT('Ctrl Pts',(-23.534,11.9528722694146,-10.9825889536698));
#116774=CARTESIAN_POINT('Ctrl Pts',(-23.534,12.007918281115,-10.9508445269094));
#116775=CARTESIAN_POINT('Ctrl Pts',(-23.534,12.0622961454218,-10.9178981000613));
#116776=CARTESIAN_POINT('Ctrl Pts',(-23.534,12.115958959572,-10.8837627538526));
#116777=CARTESIAN_POINT('Ctrl Pts',(-23.534,12.1331643569177,-10.8728182626933));
#116778=CARTESIAN_POINT('Ctrl Pts',(-23.534,12.150294211089,-10.8617527782972));
#116779=CARTESIAN_POINT('Ctrl Pts',(-23.534,12.1673397958196,-10.8505716388401));
#116780=CARTESIAN_POINT('Ctrl Pts',(-23.534,12.2766355142431,-10.7788785471058));
#116781=CARTESIAN_POINT('Ctrl Pts',(-23.534,12.3825568873877,-10.7023781389818));
#116782=CARTESIAN_POINT('Ctrl Pts',(-23.534,12.4847306195173,-10.6212230158632));
#116783=CARTESIAN_POINT('Ctrl Pts',(-23.534,12.5574317395048,-10.5634775638721));
#116784=CARTESIAN_POINT('Ctrl Pts',(-23.534,12.6282347834107,-10.503374641833));
#116785=CARTESIAN_POINT('Ctrl Pts',(-23.534,12.6969925515033,-10.4409593113222));
#116786=CARTESIAN_POINT('Ctrl Pts',(-23.534,12.7737176242397,-10.3713116059626));
#116787=CARTESIAN_POINT('Ctrl Pts',(-23.534,12.8478962945781,-10.2987843938166));
#116788=CARTESIAN_POINT('Ctrl Pts',(-23.534,12.9193848394627,-10.2235362295063));
#116789=CARTESIAN_POINT('Ctrl Pts',(23.5308797445685,7.34306041656048,-3.78088480443338));
#116790=CARTESIAN_POINT('Ctrl Pts',(23.492093981254,7.86605497010199,-3.32818419228394));
#116791=CARTESIAN_POINT('Ctrl Pts',(23.4145263363035,9.13628619196831,-2.68291557707719));
#116792=CARTESIAN_POINT('Ctrl Pts',(23.2981768097169,11.273827201379,-2.72051676872855));
#116793=CARTESIAN_POINT('Ctrl Pts',(23.1818311648087,13.1445058509814,-3.7545693255618));
#116794=CARTESIAN_POINT('Ctrl Pts',(23.0654855199005,14.3133278040104,-5.54430636416698));
#116795=CARTESIAN_POINT('Ctrl Pts',(22.9491398749923,14.5078915515634,-7.6729906495586));
#116796=CARTESIAN_POINT('Ctrl Pts',(22.8327942300841,13.683012039168,-9.64497426174501));
#116797=CARTESIAN_POINT('Ctrl Pts',(22.7164485851759,12.0307010434993,-11.0010914771052));
#116798=CARTESIAN_POINT('Ctrl Pts',(22.6001029402677,9.93571567134801,-11.4255794825061));
#116799=CARTESIAN_POINT('Ctrl Pts',(22.4837572953595,7.88584799806227,-10.819598573941));
#116800=CARTESIAN_POINT('Ctrl Pts',(22.3674116504513,6.35840201881396,-9.32424771654229));
#116801=CARTESIAN_POINT('Ctrl Pts',(22.2510660055431,5.70903363319746,-7.28771027158123));
#116802=CARTESIAN_POINT('Ctrl Pts',(22.1347203606349,6.08894046342753,-5.18418094981214));
#116803=CARTESIAN_POINT('Ctrl Pts',(22.0183747157267,7.409673761906,-3.50345455895014));
#116804=CARTESIAN_POINT('Ctrl Pts',(21.9020290708185,9.36368649127951,-2.63687572721834));
#116805=CARTESIAN_POINT('Ctrl Pts',(21.7856834259103,11.496046351416,-2.78622644534918));
#116806=CARTESIAN_POINT('Ctrl Pts',(21.6693377810021,13.3101469114119,-3.91672197416435));
#116807=CARTESIAN_POINT('Ctrl Pts',(21.5529921360939,14.3837946056831,-5.76515297562463));
#116808=CARTESIAN_POINT('Ctrl Pts',(21.4366464911858,14.4665608124293,-7.90108278347799));
#116809=CARTESIAN_POINT('Ctrl Pts',(21.3203008462775,13.5400870289091,-9.82725897609517));
#116810=CARTESIAN_POINT('Ctrl Pts',(21.2039552013694,11.8181864808081,-11.0950041454724));
#116811=CARTESIAN_POINT('Ctrl Pts',(21.0876095564611,9.70579060275323,-11.4095065743484));
#116812=CARTESIAN_POINT('Ctrl Pts',(20.971263911553,7.68639780494903,-10.6967511237975));
#116813=CARTESIAN_POINT('Ctrl Pts',(20.8549182666448,6.24770301872872,-9.12434926157139));
#116814=CARTESIAN_POINT('Ctrl Pts',(20.6997907401005,5.50261576576667,-6.36488878700103));
#116815=CARTESIAN_POINT('Ctrl Pts',(20.5058813319202,7.26494661953086,-2.90538188427047));
#116816=CARTESIAN_POINT('Ctrl Pts',(20.2731900421038,11.9254495265014,-2.33672551939335));
#116817=CARTESIAN_POINT('Ctrl Pts',(20.0792806339235,14.4679218283246,-5.27097715185977));
#116818=CARTESIAN_POINT('Ctrl Pts',(19.9241531073792,14.4082134957746,-8.1286356409495));
#116819=CARTESIAN_POINT('Ctrl Pts',(19.807807462471,13.3898163849714,-10.0008422612073));
#116820=CARTESIAN_POINT('Ctrl Pts',(19.6914618175628,11.6010543926055,-11.1782538879465));
#116821=CARTESIAN_POINT('Ctrl Pts',(19.5751161726546,9.47501136884743,-11.3809092222496));
#116822=CARTESIAN_POINT('Ctrl Pts',(19.4587705277464,7.49879745073454,-10.5643935384525));
#116823=CARTESIAN_POINT('Ctrl Pts',(19.3424248828382,6.13635193741054,-8.91750233992758));
#116824=CARTESIAN_POINT('Ctrl Pts',(19.22607923793,5.70310051443743,-6.8243373694708));
#116825=CARTESIAN_POINT('Ctrl Pts',(19.1097335930218,6.30078881484329,-4.77197647671063));
#116826=CARTESIAN_POINT('Ctrl Pts',(18.9933879481137,7.78983506549335,-3.23844387325101));
#116827=CARTESIAN_POINT('Ctrl Pts',(18.8770423032055,9.82372176647143,-2.58074401943319));
#116828=CARTESIAN_POINT('Ctrl Pts',(18.7606966582973,11.9287765236596,-2.95205128760764));
#116829=CARTESIAN_POINT('Ctrl Pts',(18.6443510133891,13.6148953672596,-4.26589332221704));
#116830=CARTESIAN_POINT('Ctrl Pts',(18.5280053684809,14.4894546634699,-6.21635758608087));
#116831=CARTESIAN_POINT('Ctrl Pts',(18.4116597235727,14.3488283537461,-8.34928709874185));
#116832=CARTESIAN_POINT('Ctrl Pts',(18.2953140786645,13.2257568308521,-10.1680437511583));
#116833=CARTESIAN_POINT('Ctrl Pts',(18.1789684337563,11.3817398772988,-11.2491412557967));
#116834=CARTESIAN_POINT('Ctrl Pts',(18.0626227888481,9.24615026099209,-11.3408514895768));
#116835=CARTESIAN_POINT('Ctrl Pts',(17.9462771439399,7.31623493710189,-10.4218235406992));
#116836=CARTESIAN_POINT('Ctrl Pts',(17.8299314990317,6.04138851298324,-8.70604028760065));
#116837=CARTESIAN_POINT('Ctrl Pts',(17.7135858541235,5.71839679930902,-6.59302628110828));
#116838=CARTESIAN_POINT('Ctrl Pts',(17.5972402092153,6.42258013691471,-4.57475245125364));
#116839=CARTESIAN_POINT('Ctrl Pts',(17.4808945643071,7.98973446887496,-3.1212289391666));
#116840=CARTESIAN_POINT('Ctrl Pts',(17.3645489193989,10.0554518264208,-2.57077253162166));
#116841=CARTESIAN_POINT('Ctrl Pts',(17.2869851561268,11.4435020078058,-2.89162900717149));
#116842=CARTESIAN_POINT('Ctrl Pts',(17.2482032744907,12.0599591502202,-3.20523048596805));
#116843=CARTESIAN_POINT('Ctrl Pts',(23.6934845769398,7.15873664017536,-3.56793941240261));
#116844=CARTESIAN_POINT('Ctrl Pts',(23.6546988136254,7.71632743320132,-3.08529252512158));
#116845=CARTESIAN_POINT('Ctrl Pts',(23.5771311686748,9.07058481414467,-2.39733920623614));
#116846=CARTESIAN_POINT('Ctrl Pts',(23.4607816420882,11.3495247734463,-2.43742772748293));
#116847=CARTESIAN_POINT('Ctrl Pts',(23.34443599718,13.343949351418,-3.53988315706783));
#116848=CARTESIAN_POINT('Ctrl Pts',(23.2280903522717,14.5900892113502,-5.44801181329597));
#116849=CARTESIAN_POINT('Ctrl Pts',(23.1117447073636,14.7975234065203,-7.71750917374831));
#116850=CARTESIAN_POINT('Ctrl Pts',(22.9953990624555,13.9180778781628,-9.81994006658924));
#116851=CARTESIAN_POINT('Ctrl Pts',(22.8790534175472,12.1564660369653,-11.2657648240908));
#116852=CARTESIAN_POINT('Ctrl Pts',(22.7627077726391,9.9228967825145,-11.718332832608));
#116853=CARTESIAN_POINT('Ctrl Pts',(22.6463621277308,7.73742977562921,-11.072266113409));
#116854=CARTESIAN_POINT('Ctrl Pts',(22.5300164828226,6.10894280744555,-9.47799736857629));
#116855=CARTESIAN_POINT('Ctrl Pts',(22.4136708379145,5.41661851716373,-7.30674238843666));
#116856=CARTESIAN_POINT('Ctrl Pts',(22.2973251930063,5.82165629300578,-5.064063999654));
#116857=CARTESIAN_POINT('Ctrl Pts',(22.180979548098,7.22975647739126,-3.27215707673417));
#116858=CARTESIAN_POINT('Ctrl Pts',(22.0646339031898,9.31302770837495,-2.34825380712489));
#116859=CARTESIAN_POINT('Ctrl Pts',(21.9482882582816,11.586443783894,-2.50748411802901));
#116860=CARTESIAN_POINT('Ctrl Pts',(21.8319426133734,13.5205476154298,-3.71276224981039));
#116861=CARTESIAN_POINT('Ctrl Pts',(21.7155969684652,14.6652174121329,-5.68346749134442));
#116862=CARTESIAN_POINT('Ctrl Pts',(21.599251323557,14.7534586271567,-7.96068966764422));
#116863=CARTESIAN_POINT('Ctrl Pts',(21.4829056786489,13.7656983375463,-10.0142829669937));
#116864=CARTESIAN_POINT('Ctrl Pts',(21.3665600337407,11.9298935750953,-11.3658898423639));
#116865=CARTESIAN_POINT('Ctrl Pts',(21.2502143888324,9.67776210478953,-11.7011966969728));
#116866=CARTESIAN_POINT('Ctrl Pts',(21.1338687439242,7.52478589512584,-10.9412922692592));
#116867=CARTESIAN_POINT('Ctrl Pts',(21.0175230990161,5.99092103680429,-9.26487557356499));
#116868=CARTESIAN_POINT('Ctrl Pts',(20.8623955724718,5.1965460486914,-6.3228759983871));
#116869=CARTESIAN_POINT('Ctrl Pts',(20.6684861642916,7.07545559310313,-2.63452172335695));
#116870=CARTESIAN_POINT('Ctrl Pts',(20.4357948744751,12.0442521019777,-2.02824857709958));
#116871=CARTESIAN_POINT('Ctrl Pts',(20.2418854662947,14.7549096746432,-5.15660179532254));
#116872=CARTESIAN_POINT('Ctrl Pts',(20.0867579397505,14.6912516187967,-8.20329521180079));
#116873=CARTESIAN_POINT('Ctrl Pts',(19.9704122948423,13.6054872474799,-10.1993488361244));
#116874=CARTESIAN_POINT('Ctrl Pts',(19.8540666499341,11.698398137079,-11.4546465791426));
#116875=CARTESIAN_POINT('Ctrl Pts',(19.7377210050259,9.43171675847363,-11.6707076218434));
#116876=CARTESIAN_POINT('Ctrl Pts',(19.6213753601177,7.32477572375777,-10.800179191741));
#116877=CARTESIAN_POINT('Ctrl Pts',(19.5050297152095,5.87220404956978,-9.0443456688206));
#116878=CARTESIAN_POINT('Ctrl Pts',(19.3886840703013,5.41029292089868,-6.81271723615754));
#116879=CARTESIAN_POINT('Ctrl Pts',(19.2723384253932,6.04751847353379,-4.62459208261562));
#116880=CARTESIAN_POINT('Ctrl Pts',(19.155992780485,7.63506556007606,-2.98961585828608));
#116881=CARTESIAN_POINT('Ctrl Pts',(19.0396471355767,9.80349444875913,-2.28840897079557));
#116882=CARTESIAN_POINT('Ctrl Pts',(18.9233014906685,12.0477991809505,-2.68427832108942));
#116883=CARTESIAN_POINT('Ctrl Pts',(18.8069558457603,13.8454552689013,-4.08503138252743));
#116884=CARTESIAN_POINT('Ctrl Pts',(18.6906102008522,14.7778669129997,-6.16451941599185));
#116885=CARTESIAN_POINT('Ctrl Pts',(18.5742645559441,14.6279381326173,-8.4385428267131));
#116886=CARTESIAN_POINT('Ctrl Pts',(18.4579189110359,13.4305751068745,-10.3776107525164));
#116887=CARTESIAN_POINT('Ctrl Pts',(18.3415732661277,11.4645759037805,-11.5302231666757));
#116888=CARTESIAN_POINT('Ctrl Pts',(18.2252276212194,9.18771642279568,-11.6280000586831));
#116889=CARTESIAN_POINT('Ctrl Pts',(18.1088819763111,7.13013664756869,-10.6481781478091));
#116890=CARTESIAN_POINT('Ctrl Pts',(17.992536331403,5.77095876742236,-8.81889534117678));
#116891=CARTESIAN_POINT('Ctrl Pts',(17.8761906864949,5.42660105939486,-6.5661048530603));
#116892=CARTESIAN_POINT('Ctrl Pts',(17.7598450415866,6.17736632643707,-4.41432163139647));
#116893=CARTESIAN_POINT('Ctrl Pts',(17.6434993966784,7.84818836623569,-2.86464712274567));
#116894=CARTESIAN_POINT('Ctrl Pts',(17.5271537517702,10.0505535185336,-2.27777786620982));
#116895=CARTESIAN_POINT('Ctrl Pts',(17.4495899884982,11.5304236169073,-2.61985908949955));
#116896=CARTESIAN_POINT('Ctrl Pts',(17.410808106862,12.1876595758245,-2.95420539592318));
#116897=CARTESIAN_POINT('Ctrl Pts',(23.8560894093112,6.97441286379024,-3.35499402037186));
#116898=CARTESIAN_POINT('Ctrl Pts',(23.8173036459966,7.56659989630065,-2.84240085795923));
#116899=CARTESIAN_POINT('Ctrl Pts',(23.7397360010461,9.00488343632105,-2.11176283539509));
#116900=CARTESIAN_POINT('Ctrl Pts',(23.6233864744595,11.4252223455135,-2.15433868623731));
#116901=CARTESIAN_POINT('Ctrl Pts',(23.5070408295513,13.5433928518545,-3.32519698857386));
#116902=CARTESIAN_POINT('Ctrl Pts',(23.3906951846431,14.8668506186901,-5.35171726242495));
#116903=CARTESIAN_POINT('Ctrl Pts',(23.2743495397349,15.0871552614771,-7.76202769793803));
#116904=CARTESIAN_POINT('Ctrl Pts',(23.1580038948267,14.1531437171576,-9.99490587143344));
#116905=CARTESIAN_POINT('Ctrl Pts',(23.0416582499186,12.2822310304315,-11.5304381710766));
#116906=CARTESIAN_POINT('Ctrl Pts',(22.9253126050104,9.91007789368101,-12.0110861827097));
#116907=CARTESIAN_POINT('Ctrl Pts',(22.8089669601021,7.58901155319615,-11.3249336528771));
#116908=CARTESIAN_POINT('Ctrl Pts',(22.692621315194,5.85948359607716,-9.63174702061027));
#116909=CARTESIAN_POINT('Ctrl Pts',(22.5762756702858,5.12420340112999,-7.32577450529211));
#116910=CARTESIAN_POINT('Ctrl Pts',(22.4599300253776,5.55437212258404,-4.94394704949586));
#116911=CARTESIAN_POINT('Ctrl Pts',(22.3435843804694,7.04983919287652,-3.0408595945182));
#116912=CARTESIAN_POINT('Ctrl Pts',(22.2272387355612,9.2623689254704,-2.05963188703145));
#116913=CARTESIAN_POINT('Ctrl Pts',(22.110893090653,11.6768412163722,-2.22874179070883));
#116914=CARTESIAN_POINT('Ctrl Pts',(21.9945474457448,13.7309483194478,-3.50880252545644));
#116915=CARTESIAN_POINT('Ctrl Pts',(21.8782018008366,14.9466402185827,-5.60178200706422));
#116916=CARTESIAN_POINT('Ctrl Pts',(21.7618561559284,15.0403564418842,-8.02029655181046));
#116917=CARTESIAN_POINT('Ctrl Pts',(21.6455105110202,13.9913096461837,-10.2013069578923));
#116918=CARTESIAN_POINT('Ctrl Pts',(21.529164866112,12.0416006693825,-11.6367755392554));
#116919=CARTESIAN_POINT('Ctrl Pts',(21.4128192212038,9.64973360682584,-11.9928868195971));
#116920=CARTESIAN_POINT('Ctrl Pts',(21.2964735762957,7.36317398530266,-11.185833414721));
#116921=CARTESIAN_POINT('Ctrl Pts',(21.1801279313874,5.73413905487985,-9.4054018855586));
#116922=CARTESIAN_POINT('Ctrl Pts',(21.0250004048432,4.89047633161614,-6.28086320977319));
#116923=CARTESIAN_POINT('Ctrl Pts',(20.8310909966629,6.88596456667538,-2.36366156244345));
#116924=CARTESIAN_POINT('Ctrl Pts',(20.5983997068464,12.1630546774541,-1.71977163480581));
#116925=CARTESIAN_POINT('Ctrl Pts',(20.4044902986661,15.0418975209619,-5.04222643878529));
#116926=CARTESIAN_POINT('Ctrl Pts',(20.2493627721219,14.9742897418189,-8.2779547826521));
#116927=CARTESIAN_POINT('Ctrl Pts',(20.1330171272137,13.8211581099884,-10.3978554110414));
#116928=CARTESIAN_POINT('Ctrl Pts',(20.0166714823055,11.7957418815525,-11.7310392703387));
#116929=CARTESIAN_POINT('Ctrl Pts',(19.9003258373973,9.38842214809981,-11.9605060214371));
#116930=CARTESIAN_POINT('Ctrl Pts',(19.7839801924891,7.15075399678101,-11.0359648450295));
#116931=CARTESIAN_POINT('Ctrl Pts',(19.6676345475809,5.60805616172902,-9.17118899771363));
#116932=CARTESIAN_POINT('Ctrl Pts',(19.5512889026727,5.11748532735993,-6.8010971028443));
#116933=CARTESIAN_POINT('Ctrl Pts',(19.4349432577645,5.79424813222429,-4.47720768852061));
#116934=CARTESIAN_POINT('Ctrl Pts',(19.3185976128563,7.48029605465876,-2.74078784332114));
#116935=CARTESIAN_POINT('Ctrl Pts',(19.2022519679481,9.78326713104683,-1.99607392215794));
#116936=CARTESIAN_POINT('Ctrl Pts',(19.0859063230399,12.1668218382416,-2.41650535457117));
#116937=CARTESIAN_POINT('Ctrl Pts',(18.9695606781317,14.0760151705431,-3.90416944283784));
#116938=CARTESIAN_POINT('Ctrl Pts',(18.8532150332235,15.0662791625295,-6.11268124590282));
#116939=CARTESIAN_POINT('Ctrl Pts',(18.7368693883153,14.9070479114883,-8.52779855468437));
#116940=CARTESIAN_POINT('Ctrl Pts',(18.6205237434071,13.6353933828971,-10.5871777538744));
#116941=CARTESIAN_POINT('Ctrl Pts',(18.504178098499,11.5474119302623,-11.8113050775549));
#116942=CARTESIAN_POINT('Ctrl Pts',(18.3878324535907,9.12928258459928,-11.9151486277894));
#116943=CARTESIAN_POINT('Ctrl Pts',(18.2714868086826,6.94403835803548,-10.8745327549191));
#116944=CARTESIAN_POINT('Ctrl Pts',(18.1551411637744,5.50052902186147,-8.93175039475289));
#116945=CARTESIAN_POINT('Ctrl Pts',(18.0387955188662,5.13480531948069,-6.53918342501231));
#116946=CARTESIAN_POINT('Ctrl Pts',(17.922449873958,5.93215251595945,-4.2538908115393));
#116947=CARTESIAN_POINT('Ctrl Pts',(17.8061042290498,7.70664226359641,-2.60806530632473));
#116948=CARTESIAN_POINT('Ctrl Pts',(17.6897585841416,10.0456552106465,-1.98478320079797));
#116949=CARTESIAN_POINT('Ctrl Pts',(17.6121948208694,11.6173452260086,-2.34808917182759));
#116950=CARTESIAN_POINT('Ctrl Pts',(17.5734129392334,12.3153600014288,-2.70318030587831));
#116951=CARTESIAN_POINT('Ctrl Pts',(24.0186942416826,6.79008908740512,-3.14204862834109));
#116952=CARTESIAN_POINT('Ctrl Pts',(23.979908478368,7.41687235939997,-2.59950919079688));
#116953=CARTESIAN_POINT('Ctrl Pts',(23.9023408334175,8.93918205849745,-1.82618646455404));
#116954=CARTESIAN_POINT('Ctrl Pts',(23.7859913068309,11.5009199175807,-1.87124964499168));
#116955=CARTESIAN_POINT('Ctrl Pts',(23.6696456619227,13.7428363522911,-3.11051082007989));
#116956=CARTESIAN_POINT('Ctrl Pts',(23.5533000170145,15.14361202603,-5.25542271155395));
#116957=CARTESIAN_POINT('Ctrl Pts',(23.4369543721063,15.3767871164341,-7.80654622212773));
#116958=CARTESIAN_POINT('Ctrl Pts',(23.3206087271981,14.3882095561523,-10.1698716762777));
#116959=CARTESIAN_POINT('Ctrl Pts',(23.2042630822899,12.4079960238977,-11.7951115180623));
#116960=CARTESIAN_POINT('Ctrl Pts',(23.0879174373818,9.89725900484749,-12.3038395328114));
#116961=CARTESIAN_POINT('Ctrl Pts',(22.9715717924735,7.4405933307631,-11.5776011923451));
#116962=CARTESIAN_POINT('Ctrl Pts',(22.8552261475653,5.61002438470876,-9.78549667264426));
#116963=CARTESIAN_POINT('Ctrl Pts',(22.7388805026571,4.83178828509627,-7.34480662214755));
#116964=CARTESIAN_POINT('Ctrl Pts',(22.622534857749,5.28708795216229,-4.82383009933772));
#116965=CARTESIAN_POINT('Ctrl Pts',(22.5061892128408,6.86992190836178,-2.80956211230224));
#116966=CARTESIAN_POINT('Ctrl Pts',(22.3898435679325,9.21171014256585,-1.771009966938));
#116967=CARTESIAN_POINT('Ctrl Pts',(22.2734979230244,11.7672386488503,-1.94999946338866));
#116968=CARTESIAN_POINT('Ctrl Pts',(22.1571522781162,13.9413490234657,-3.30484280110248));
#116969=CARTESIAN_POINT('Ctrl Pts',(22.040806633208,15.2280630250325,-5.52009652278402));
#116970=CARTESIAN_POINT('Ctrl Pts',(21.9244609882998,15.3272542566116,-8.07990343597667));
#116971=CARTESIAN_POINT('Ctrl Pts',(21.8081153433916,14.216920954821,-10.3883309487909));
#116972=CARTESIAN_POINT('Ctrl Pts',(21.6917696984834,12.1533077636698,-11.907661236147));
#116973=CARTESIAN_POINT('Ctrl Pts',(21.5754240535752,9.62170510886214,-12.2845769422216));
#116974=CARTESIAN_POINT('Ctrl Pts',(21.459078408667,7.20156207547948,-11.4303745601828));
#116975=CARTESIAN_POINT('Ctrl Pts',(21.3427327637588,5.47735707295543,-9.54592819755221));
#116976=CARTESIAN_POINT('Ctrl Pts',(21.1876052372145,4.58440661454088,-6.23885042115928));
#116977=CARTESIAN_POINT('Ctrl Pts',(20.9936958290342,6.69647354024763,-2.09280140152994));
#116978=CARTESIAN_POINT('Ctrl Pts',(20.7610045392178,12.2818572529304,-1.41129469251204));
#116979=CARTESIAN_POINT('Ctrl Pts',(20.5670951310375,15.3288853672806,-4.92785108224806));
#116980=CARTESIAN_POINT('Ctrl Pts',(20.4119676044933,15.257327864841,-8.35261435350337));
#116981=CARTESIAN_POINT('Ctrl Pts',(20.295621959585,14.0368289724969,-10.5963619859584));
#116982=CARTESIAN_POINT('Ctrl Pts',(20.1792763146769,11.893085626026,-12.0074319615348));
#116983=CARTESIAN_POINT('Ctrl Pts',(20.0629306697686,9.345127537726,-12.2503044210308));
#116984=CARTESIAN_POINT('Ctrl Pts',(19.9465850248605,6.97673226980424,-11.2717504983181));
#116985=CARTESIAN_POINT('Ctrl Pts',(19.8302393799522,5.34390827388827,-9.29803232660665));
#116986=CARTESIAN_POINT('Ctrl Pts',(19.7138937350441,4.82467773382117,-6.78947696953105));
#116987=CARTESIAN_POINT('Ctrl Pts',(19.5975480901359,5.54097779091479,-4.3298232944256));
#116988=CARTESIAN_POINT('Ctrl Pts',(19.4812024452277,7.32552654924147,-2.49195982835622));
#116989=CARTESIAN_POINT('Ctrl Pts',(19.3648568003195,9.76303981333453,-1.70373887352032));
#116990=CARTESIAN_POINT('Ctrl Pts',(19.2485111554113,12.2858444955327,-2.14873238805294));
#116991=CARTESIAN_POINT('Ctrl Pts',(19.1321655105031,14.3065750721849,-3.72330750314826));
#116992=CARTESIAN_POINT('Ctrl Pts',(19.0158198655949,15.3546914120593,-6.0608430758138));
#116993=CARTESIAN_POINT('Ctrl Pts',(18.8994742206867,15.1861576903593,-8.61705428265562));
#116994=CARTESIAN_POINT('Ctrl Pts',(18.7831285757785,13.8402116589195,-10.7967447552324));
#116995=CARTESIAN_POINT('Ctrl Pts',(18.6667829308703,11.6302479567442,-12.0923869884339));
#116996=CARTESIAN_POINT('Ctrl Pts',(18.5504372859621,9.07084874640288,-12.2022971968956));
#116997=CARTESIAN_POINT('Ctrl Pts',(18.4340916410539,6.75794006850229,-11.1008873620291));
#116998=CARTESIAN_POINT('Ctrl Pts',(18.3177459961457,5.23009927630059,-9.04460544832903));
#116999=CARTESIAN_POINT('Ctrl Pts',(18.2014003512375,4.84300957956654,-6.51226199696434));
#117000=CARTESIAN_POINT('Ctrl Pts',(18.0850547063294,5.68693870548182,-4.09345999168212));
#117001=CARTESIAN_POINT('Ctrl Pts',(17.9687090614211,7.56509616095713,-2.35148348990379));
#117002=CARTESIAN_POINT('Ctrl Pts',(17.852363416513,10.0407569027593,-1.69178853538612));
#117003=CARTESIAN_POINT('Ctrl Pts',(17.7747996532408,11.70426683511,-2.07631925415564));
#117004=CARTESIAN_POINT('Ctrl Pts',(17.7360177716048,12.4430604270331,-2.45215521583344));
#117005=CARTESIAN_POINT('Ctrl Pts',(17.734,12.4414757859805,-2.45527019889633));
#117006=CARTESIAN_POINT('Ctrl Pts',(17.734,12.3039867051776,-2.39880617496762));
#117007=CARTESIAN_POINT('Ctrl Pts',(17.734,12.1641669931158,-2.34855999836891));
#117008=CARTESIAN_POINT('Ctrl Pts',(17.734,12.0224504771058,-2.30458254792745));
#117009=CARTESIAN_POINT('Ctrl Pts',(17.734,11.8806702982859,-2.26058534165126));
#117010=CARTESIAN_POINT('Ctrl Pts',(17.734,11.7369908080183,-2.22286244827998));
#117011=CARTESIAN_POINT('Ctrl Pts',(17.734,11.5918412576186,-2.19151632697145));
#117012=CARTESIAN_POINT('Ctrl Pts',(17.734,11.5283759217618,-2.1778105172657));
#117013=CARTESIAN_POINT('Ctrl Pts',(17.734,11.4646295457121,-2.16532448472317));
#117014=CARTESIAN_POINT('Ctrl Pts',(17.734,11.4006382986832,-2.15406992347917));
#117015=CARTESIAN_POINT('Ctrl Pts',(17.734,11.3633072808146,-2.14750427198133));
#117016=CARTESIAN_POINT('Ctrl Pts',(17.734,11.325892119771,-2.14135763815236));
#117017=CARTESIAN_POINT('Ctrl Pts',(17.734,11.2884026214455,-2.13563303349493));
#117018=CARTESIAN_POINT('Ctrl Pts',(17.734,11.2692561047234,-2.13270938170717));
#117019=CARTESIAN_POINT('Ctrl Pts',(17.734,11.250091584631,-2.12989604625388));
#117020=CARTESIAN_POINT('Ctrl Pts',(17.734,11.2309171197761,-2.12719424914615));
#117021=CARTESIAN_POINT('Ctrl Pts',(17.734,11.0859964654593,-2.10677405970945));
#117022=CARTESIAN_POINT('Ctrl Pts',(17.734,10.9403799749511,-2.09270150463882));
#117023=CARTESIAN_POINT('Ctrl Pts',(17.734,10.7944837770183,-2.0850637244268));
#117024=CARTESIAN_POINT('Ctrl Pts',(17.734,10.6507966464811,-2.07754159062285));
#117025=CARTESIAN_POINT('Ctrl Pts',(17.734,10.5068375056605,-2.07626094200616));
#117026=CARTESIAN_POINT('Ctrl Pts',(17.734,10.3630121887439,-2.08135439022795));
#117027=CARTESIAN_POINT('Ctrl Pts',(17.734,10.2786127987136,-2.08434332105241));
#117028=CARTESIAN_POINT('Ctrl Pts',(17.734,10.19425970219,-2.08952813543896));
#117029=CARTESIAN_POINT('Ctrl Pts',(17.734,10.1100377343263,-2.0969435515888));
#117030=CARTESIAN_POINT('Ctrl Pts',(17.734,10.0914524803675,-2.09857991079354));
#117031=CARTESIAN_POINT('Ctrl Pts',(17.734,10.0728758846397,-2.10032474830959));
#117032=CARTESIAN_POINT('Ctrl Pts',(17.734,10.054317787698,-2.10217740077462));
#117033=CARTESIAN_POINT('Ctrl Pts',(17.734,10.0520311372889,-2.10240567679508));
#117034=CARTESIAN_POINT('Ctrl Pts',(17.734,10.0497447287136,-2.1026355930538));
#117035=CARTESIAN_POINT('Ctrl Pts',(17.734,10.0474585635589,-2.10286714977861));
#117036=CARTESIAN_POINT('Ctrl Pts',(17.734,9.90553857679407,-2.11724167003299));
#117037=CARTESIAN_POINT('Ctrl Pts',(17.734,9.76455596495627,-2.13793360360503));
#117038=CARTESIAN_POINT('Ctrl Pts',(17.734,9.62489441371198,-2.164760150274));
#117039=CARTESIAN_POINT('Ctrl Pts',(17.734,9.48423704389368,-2.19177797631236));
#117040=CARTESIAN_POINT('Ctrl Pts',(17.734,9.34491888121941,-2.2250185138435));
#117041=CARTESIAN_POINT('Ctrl Pts',(17.734,9.20734701484862,-2.26434539663517));
#117042=CARTESIAN_POINT('Ctrl Pts',(17.734,9.07102557836913,-2.30331482618387));
#117043=CARTESIAN_POINT('Ctrl Pts',(17.734,8.93641816462683,-2.34826086893132));
#117044=CARTESIAN_POINT('Ctrl Pts',(17.734,8.80394629780779,-2.39909462202466));
#117045=CARTESIAN_POINT('Ctrl Pts',(17.734,8.6733123432917,-2.44922310853983));
#117046=CARTESIAN_POINT('Ctrl Pts',(17.734,8.54475450722417,-2.50507746121123));
#117047=CARTESIAN_POINT('Ctrl Pts',(17.734,8.41871108205256,-2.56660923674854));
#117048=CARTESIAN_POINT('Ctrl Pts',(17.734,8.3906008252741,-2.58033207876138));
#117049=CARTESIAN_POINT('Ctrl Pts',(17.734,8.36261639474796,-2.5943371237179));
#117050=CARTESIAN_POINT('Ctrl Pts',(17.734,8.33476077836578,-2.60862517191624));
#117051=CARTESIAN_POINT('Ctrl Pts',(17.734,8.31199476146196,-2.6203025996329));
#117052=CARTESIAN_POINT('Ctrl Pts',(17.734,8.28931855882506,-2.63216728051035));
#117053=CARTESIAN_POINT('Ctrl Pts',(17.734,8.2667549368276,-2.64420787330719));
#117054=CARTESIAN_POINT('Ctrl Pts',(17.734,8.14790051039562,-2.70763198805837));
#117055=CARTESIAN_POINT('Ctrl Pts',(17.734,8.0320302386953,-2.77600356607502));
#117056=CARTESIAN_POINT('Ctrl Pts',(17.734,7.91948448293877,-2.84921041197833));
#117057=CARTESIAN_POINT('Ctrl Pts',(17.734,7.89990776773299,-2.86194434018138));
#117058=CARTESIAN_POINT('Ctrl Pts',(17.734,7.88043170399221,-2.87482465916843));
#117059=CARTESIAN_POINT('Ctrl Pts',(17.734,7.86105816656312,-2.88785089183458));
#117060=CARTESIAN_POINT('Ctrl Pts',(17.734,7.74528165055071,-2.96569583060086));
#117061=CARTESIAN_POINT('Ctrl Pts',(17.734,7.63316351668275,-3.04874885969153));
#117062=CARTESIAN_POINT('Ctrl Pts',(17.734,7.52499462458606,-3.13669681545413));
#117063=CARTESIAN_POINT('Ctrl Pts',(17.734,7.41763480850288,-3.2239869427037));
#117064=CARTESIAN_POINT('Ctrl Pts',(17.734,7.31416494711279,-3.31609973202711));
#117065=CARTESIAN_POINT('Ctrl Pts',(17.734,7.214911090176,-3.41275797650577));
#117066=CARTESIAN_POINT('Ctrl Pts',(17.734,7.13012408682151,-3.49532769371153));
#117067=CARTESIAN_POINT('Ctrl Pts',(17.734,7.04841415790898,-3.58121506916121));
#117068=CARTESIAN_POINT('Ctrl Pts',(17.734,6.9700124957236,-3.67025869427777));
#117069=CARTESIAN_POINT('Ctrl Pts',(17.734,6.95431915067657,-3.68808219819647));
#117070=CARTESIAN_POINT('Ctrl Pts',(17.734,6.93875844510523,-3.70603218668507));
#117071=CARTESIAN_POINT('Ctrl Pts',(17.734,6.92333236973455,-3.72410739902025));
#117072=CARTESIAN_POINT('Ctrl Pts',(17.734,6.91090397970631,-3.7386701301976));
#117073=CARTESIAN_POINT('Ctrl Pts',(17.734,6.89856246392884,-3.75331485694984));
#117074=CARTESIAN_POINT('Ctrl Pts',(17.734,6.88631933290202,-3.7680280979283));
#117075=CARTESIAN_POINT('Ctrl Pts',(17.734,6.79919924774975,-3.87272507487817));
#117076=CARTESIAN_POINT('Ctrl Pts',(17.734,6.71692866786336,-3.98103806042148));
#117077=CARTESIAN_POINT('Ctrl Pts',(17.734,6.63977277908297,-4.09267000357134));
#117078=CARTESIAN_POINT('Ctrl Pts',(17.734,6.5632613323866,-4.20336954449987));
#117079=CARTESIAN_POINT('Ctrl Pts',(17.734,6.49177912370978,-4.31733350190904));
#117080=CARTESIAN_POINT('Ctrl Pts',(17.734,6.42562994043966,-4.43429573639373));
#117081=CARTESIAN_POINT('Ctrl Pts',(17.734,6.40600466641057,-4.46899632964889));
#117082=CARTESIAN_POINT('Ctrl Pts',(17.734,6.38684913115103,-4.5039609540058));
#117083=CARTESIAN_POINT('Ctrl Pts',(17.734,6.36817211518176,-4.5391829311905));
#117084=CARTESIAN_POINT('Ctrl Pts',(17.734,6.30473751328735,-4.6588108259421));
#117085=CARTESIAN_POINT('Ctrl Pts',(17.734,6.24681897356681,-4.78140717330271));
#117086=CARTESIAN_POINT('Ctrl Pts',(17.734,6.19457219597222,-4.90656879650459));
#117087=CARTESIAN_POINT('Ctrl Pts',(17.734,6.16656485885406,-4.97366276739923));
#117088=CARTESIAN_POINT('Ctrl Pts',(17.734,6.14018823211245,-5.04149397277722));
#117089=CARTESIAN_POINT('Ctrl Pts',(17.734,6.11547251223002,-5.11000011542525));
#117090=CARTESIAN_POINT('Ctrl Pts',(17.734,6.10242953315656,-5.14615217529696));
#117091=CARTESIAN_POINT('Ctrl Pts',(17.734,6.08984917083384,-5.1824921894001));
#117092=CARTESIAN_POINT('Ctrl Pts',(17.734,6.07773636071827,-5.2190109187711));
#117093=CARTESIAN_POINT('Ctrl Pts',(17.734,6.06903436379304,-5.24524643866015));
#117094=CARTESIAN_POINT('Ctrl Pts',(17.734,6.06057221982836,-5.27157936590157));
#117095=CARTESIAN_POINT('Ctrl Pts',(17.734,6.05236276271083,-5.29796985459013));
#117096=CARTESIAN_POINT('Ctrl Pts',(17.734,6.01297460247702,-5.42458879933058));
#117097=CARTESIAN_POINT('Ctrl Pts',(17.734,5.97934462682723,-5.55268880308997));
#117098=CARTESIAN_POINT('Ctrl Pts',(17.734,5.95155790702637,-5.68187791684614));
#117099=CARTESIAN_POINT('Ctrl Pts',(17.734,5.92387819466037,-5.81056951971318));
#117100=CARTESIAN_POINT('Ctrl Pts',(17.734,5.90199676488022,-5.9403426690094));
#117101=CARTESIAN_POINT('Ctrl Pts',(17.734,5.88604904275158,-6.07081358829993));
#117102=CARTESIAN_POINT('Ctrl Pts',(17.734,5.87037715516175,-6.19902786017957));
#117103=CARTESIAN_POINT('Ctrl Pts',(17.734,5.86043554854223,-6.32791668515105));
#117104=CARTESIAN_POINT('Ctrl Pts',(17.734,5.85640219965433,-6.45710818642194));
#117105=CARTESIAN_POINT('Ctrl Pts',(17.734,5.85485839225762,-6.50655761437785));
#117106=CARTESIAN_POINT('Ctrl Pts',(17.734,5.85418069613612,-6.55605124999239));
#117107=CARTESIAN_POINT('Ctrl Pts',(17.734,5.85438103290403,-6.60556760587704));
#117108=CARTESIAN_POINT('Ctrl Pts',(17.734,5.85480000921424,-6.70912413372275));
#117109=CARTESIAN_POINT('Ctrl Pts',(17.734,5.85905829450831,-6.81278078385137));
#117110=CARTESIAN_POINT('Ctrl Pts',(17.734,5.86714838588205,-6.9163217216595));
#117111=CARTESIAN_POINT('Ctrl Pts',(23.534,7.33966741897454,-3.77664721604216));
#117112=CARTESIAN_POINT('Ctrl Pts',(23.534,7.42781106532914,-3.68403366522651));
#117113=CARTESIAN_POINT('Ctrl Pts',(23.534,7.52001976376119,-3.59567730315303));
#117114=CARTESIAN_POINT('Ctrl Pts',(23.534,7.61588000351054,-3.5116960194841));
#117115=CARTESIAN_POINT('Ctrl Pts',(23.534,7.71428950783776,-3.42548137491161));
#117116=CARTESIAN_POINT('Ctrl Pts',(23.534,7.81654770306906,-3.34387704110181));
#117117=CARTESIAN_POINT('Ctrl Pts',(23.534,7.92225677096286,-3.26703375166838));
#117118=CARTESIAN_POINT('Ctrl Pts',(23.534,8.0288784923947,-3.18952702530023));
#117119=CARTESIAN_POINT('Ctrl Pts',(23.534,8.13901148194131,-3.11686336121957));
#117120=CARTESIAN_POINT('Ctrl Pts',(23.534,8.25229019245111,-3.04922905261281));
#117121=CARTESIAN_POINT('Ctrl Pts',(23.534,8.36548868721879,-2.98164263770322));
#117122=CARTESIAN_POINT('Ctrl Pts',(23.534,8.48182908276737,-2.91907793776718));
#117123=CARTESIAN_POINT('Ctrl Pts',(23.534,8.60098002351534,-2.86176024172565));
#117124=CARTESIAN_POINT('Ctrl Pts',(23.534,8.62551775116567,-2.84995633983295));
#117125=CARTESIAN_POINT('Ctrl Pts',(23.534,8.6501747700182,-2.83837511497645));
#117126=CARTESIAN_POINT('Ctrl Pts',(23.534,8.67494832377365,-2.82701877421198));
#117127=CARTESIAN_POINT('Ctrl Pts',(23.534,8.69677888932777,-2.81701151631264));
#117128=CARTESIAN_POINT('Ctrl Pts',(23.534,8.7187040887079,-2.80717716259871));
#117129=CARTESIAN_POINT('Ctrl Pts',(23.534,8.7406954034996,-2.7975286977491));
#117130=CARTESIAN_POINT('Ctrl Pts',(23.534,8.86780597067235,-2.74176023410807));
#117131=CARTESIAN_POINT('Ctrl Pts',(23.534,8.99727639743939,-2.69212556532351));
#117132=CARTESIAN_POINT('Ctrl Pts',(23.534,9.12866759232672,-2.6487952833054));
#117133=CARTESIAN_POINT('Ctrl Pts',(23.534,9.25547643309883,-2.60697617329764));
#117134=CARTESIAN_POINT('Ctrl Pts',(23.534,9.38407515938093,-2.57102868262552));
#117135=CARTESIAN_POINT('Ctrl Pts',(23.534,9.51404078368103,-2.54089289360577));
#117136=CARTESIAN_POINT('Ctrl Pts',(23.534,9.64599296324263,-2.51029647193366));
#117137=CARTESIAN_POINT('Ctrl Pts',(23.534,9.77935483569702,-2.48569051020119));
#117138=CARTESIAN_POINT('Ctrl Pts',(23.534,9.91370948271991,-2.46705966806736));
#117139=CARTESIAN_POINT('Ctrl Pts',(23.534,10.0310062349449,-2.45079422937997));
#117140=CARTESIAN_POINT('Ctrl Pts',(23.534,10.1490603917629,-2.43908365615736));
#117141=CARTESIAN_POINT('Ctrl Pts',(23.534,10.2676037380491,-2.43194887296395));
#117142=CARTESIAN_POINT('Ctrl Pts',(23.534,10.3041175791359,-2.42975120984852));
#117143=CARTESIAN_POINT('Ctrl Pts',(23.534,10.3406773911112,-2.4279879127063));
#117144=CARTESIAN_POINT('Ctrl Pts',(23.534,10.3772769926609,-2.42666011382119));
#117145=CARTESIAN_POINT('Ctrl Pts',(23.534,10.4011419710669,-2.42579431500428));
#117146=CARTESIAN_POINT('Ctrl Pts',(23.534,10.4250202863045,-2.42511392850644));
#117147=CARTESIAN_POINT('Ctrl Pts',(23.534,10.4488889853955,-2.42461930902246));
#117148=CARTESIAN_POINT('Ctrl Pts',(23.534,10.5881947642429,-2.42173254287793));
#117149=CARTESIAN_POINT('Ctrl Pts',(23.534,10.7273545089995,-2.42516221226969));
#117150=CARTESIAN_POINT('Ctrl Pts',(23.534,10.8659190931826,-2.43484421425681));
#117151=CARTESIAN_POINT('Ctrl Pts',(23.534,10.9998137686292,-2.44419991305517));
#117152=CARTESIAN_POINT('Ctrl Pts',(23.534,11.1331535299474,-2.45939375404953));
#117153=CARTESIAN_POINT('Ctrl Pts',(23.534,11.2655490821966,-2.48041129060109));
#117154=CARTESIAN_POINT('Ctrl Pts',(23.534,11.2886886126467,-2.48408464607836));
#117155=CARTESIAN_POINT('Ctrl Pts',(23.534,11.3117993244444,-2.48793600302252));
#117156=CARTESIAN_POINT('Ctrl Pts',(23.534,11.3348791639493,-2.49196542192025));
#117157=CARTESIAN_POINT('Ctrl Pts',(23.534,11.4716128752646,-2.51583722571738));
#117158=CARTESIAN_POINT('Ctrl Pts',(23.534,11.6072631372987,-2.54595436303442));
#117159=CARTESIAN_POINT('Ctrl Pts',(23.534,11.741474161821,-2.58210348353803));
#117160=CARTESIAN_POINT('Ctrl Pts',(23.534,11.8669921985643,-2.61591118787352));
#117161=CARTESIAN_POINT('Ctrl Pts',(23.534,11.9912519180839,-2.65499542884546));
#117162=CARTESIAN_POINT('Ctrl Pts',(23.534,12.1139562411199,-2.69922248208064));
#117163=CARTESIAN_POINT('Ctrl Pts',(23.534,12.1324792825538,-2.70589885271947));
#117164=CARTESIAN_POINT('Ctrl Pts',(23.534,12.1509668598302,-2.71269248793648));
#117165=CARTESIAN_POINT('Ctrl Pts',(23.534,12.1694179272643,-2.71960300224709));
#117166=CARTESIAN_POINT('Ctrl Pts',(23.534,12.1864042738565,-2.725964931801));
#117167=CARTESIAN_POINT('Ctrl Pts',(23.534,12.2033501584913,-2.73242235622137));
#117168=CARTESIAN_POINT('Ctrl Pts',(23.534,12.2202547019028,-2.73897459134067));
#117169=CARTESIAN_POINT('Ctrl Pts',(23.534,12.3523840941254,-2.79018821024404));
#117170=CARTESIAN_POINT('Ctrl Pts',(23.534,12.4819900441372,-2.84719066756166));
#117171=CARTESIAN_POINT('Ctrl Pts',(23.534,12.6087145787098,-2.90970780354203));
#117172=CARTESIAN_POINT('Ctrl Pts',(23.534,12.7371473048454,-2.97306764330177));
#117173=CARTESIAN_POINT('Ctrl Pts',(23.534,12.8626211666375,-3.04209197613929));
#117174=CARTESIAN_POINT('Ctrl Pts',(23.534,12.9847605797071,-3.11654906624453));
#117175=CARTESIAN_POINT('Ctrl Pts',(23.534,13.1066107532543,-3.19082983379632));
#117176=CARTESIAN_POINT('Ctrl Pts',(23.534,13.2251430159563,-3.27051793770692));
#117177=CARTESIAN_POINT('Ctrl Pts',(23.534,13.339970121412,-3.35543295399967));
#117178=CARTESIAN_POINT('Ctrl Pts',(23.534,13.3745616920472,-3.38101353249137));
#117179=CARTESIAN_POINT('Ctrl Pts',(23.534,13.4088168737746,-3.40706878536305));
#117180=CARTESIAN_POINT('Ctrl Pts',(23.534,13.442724662023,-3.43359460806598));
#117181=CARTESIAN_POINT('Ctrl Pts',(23.534,13.5222654936816,-3.49581883757828));
#117182=CARTESIAN_POINT('Ctrl Pts',(23.534,13.5998952497886,-3.56063180043892));
#117183=CARTESIAN_POINT('Ctrl Pts',(23.534,13.6755304223662,-3.62791906475953));
#117184=CARTESIAN_POINT('Ctrl Pts',(23.534,13.6988785584492,-3.64869025031349));
#117185=CARTESIAN_POINT('Ctrl Pts',(23.534,13.7220365683719,-3.66969729110703));
#117186=CARTESIAN_POINT('Ctrl Pts',(23.534,13.7450018328666,-3.69093701222324));
#117187=CARTESIAN_POINT('Ctrl Pts',(23.534,13.7616807918054,-3.70636276255376));
#117188=CARTESIAN_POINT('Ctrl Pts',(23.534,13.778252633284,-3.72190625726443));
#117189=CARTESIAN_POINT('Ctrl Pts',(23.534,13.794710755701,-3.73756042625356));
#117190=CARTESIAN_POINT('Ctrl Pts',(23.534,13.8994714966307,-3.83720376954566));
#117191=CARTESIAN_POINT('Ctrl Pts',(23.534,13.9997005890966,-3.94139578034812));
#117192=CARTESIAN_POINT('Ctrl Pts',(23.534,14.0951974348198,-4.04973935219095));
#117193=CARTESIAN_POINT('Ctrl Pts',(23.534,14.1919272854663,-4.15948179911159));
#117194=CARTESIAN_POINT('Ctrl Pts',(23.5339999999999,14.2838024902753,-4.27348416760674));
#117195=CARTESIAN_POINT('Ctrl Pts',(23.534,14.3705861834528,-4.39137862116285));
#117196=CARTESIAN_POINT('Ctrl Pts',(23.534,14.3939765840125,-4.42315415861089));
#117197=CARTESIAN_POINT('Ctrl Pts',(23.534,14.4169969315181,-4.45521265895928));
#117198=CARTESIAN_POINT('Ctrl Pts',(23.5339999999999,14.4396421540893,-4.48754739858326));
#117199=CARTESIAN_POINT('Ctrl Pts',(23.5339999999999,14.4633057306723,-4.52133622909603));
#117200=CARTESIAN_POINT('Ctrl Pts',(23.534,14.486559687685,-4.55542670188665));
#117201=CARTESIAN_POINT('Ctrl Pts',(23.534,14.5093979973546,-4.58981135573279));
#117202=CARTESIAN_POINT('Ctrl Pts',(23.534,14.5229724195575,-4.6102485866559));
#117203=CARTESIAN_POINT('Ctrl Pts',(23.534,14.5363970207432,-4.63078533674386));
#117204=CARTESIAN_POINT('Ctrl Pts',(23.534,14.5496664278029,-4.65141310427564));
#117205=CARTESIAN_POINT('Ctrl Pts',(23.534,14.6302131840669,-4.77662591568344));
#117206=CARTESIAN_POINT('Ctrl Pts',(23.5339999999999,14.7050940684627,-4.90526377791117));
#117207=CARTESIAN_POINT('Ctrl Pts',(23.5339999999999,14.7740779860328,-5.03693509762848));
#117208=CARTESIAN_POINT('Ctrl Pts',(23.5339999999999,14.825130242171,-5.1343798090488));
#117209=CARTESIAN_POINT('Ctrl Pts',(23.534,14.8729522304357,-5.23348688766521));
#117210=CARTESIAN_POINT('Ctrl Pts',(23.534,14.917437260214,-5.33411057035729));
#117211=CARTESIAN_POINT('Ctrl Pts',(23.534,14.9671573568045,-5.44657580299122));
#117212=CARTESIAN_POINT('Ctrl Pts',(23.5339999999999,15.012709422787,-5.56093556570213));
#117213=CARTESIAN_POINT('Ctrl Pts',(23.5339999999999,15.0540735698273,-5.67694764394986));
#117214=CARTESIAN_POINT('Ctrl Pts',(23.531982455913,15.0572810292372,-8.32379157603815));
#117215=CARTESIAN_POINT('Ctrl Pts',(23.4932005742769,14.8422321918575,-9.12430549407578));
#117216=CARTESIAN_POINT('Ctrl Pts',(23.4156368110048,14.0148884746517,-10.6178353680082));
#117217=CARTESIAN_POINT('Ctrl Pts',(23.2992911660966,11.8680998485746,-12.016187756466));
#117218=CARTESIAN_POINT('Ctrl Pts',(23.1829455211884,9.31682643229098,-12.2463209197506));
#117219=CARTESIAN_POINT('Ctrl Pts',(23.0665998762802,6.95460769844995,-11.2549881116262));
#117220=CARTESIAN_POINT('Ctrl Pts',(22.950254231372,5.33172340411622,-9.27285604389766));
#117221=CARTESIAN_POINT('Ctrl Pts',(22.8339085864638,4.82593323769868,-6.76152808689128));
#117222=CARTESIAN_POINT('Ctrl Pts',(22.7175629415556,5.55506413782101,-4.30571512371993));
#117223=CARTESIAN_POINT('Ctrl Pts',(22.6012172966474,7.34931555885556,-2.4772552638758));
#117224=CARTESIAN_POINT('Ctrl Pts',(22.4848716517392,9.79091954839253,-1.70188610485324));
#117225=CARTESIAN_POINT('Ctrl Pts',(22.368526006831,12.3113587413642,-2.16015085039805));
#117226=CARTESIAN_POINT('Ctrl Pts',(22.2521803619228,14.3237647967067,-3.74534492265297));
#117227=CARTESIAN_POINT('Ctrl Pts',(22.1358347170146,15.359565457441,-6.08836358180601));
#117228=CARTESIAN_POINT('Ctrl Pts',(22.0194890721064,15.1775701554181,-8.64365525823664));
#117229=CARTESIAN_POINT('Ctrl Pts',(21.9031434271982,13.820179034717,-10.8162231363412));
#117230=CARTESIAN_POINT('Ctrl Pts',(21.78679778229,11.6034021905309,-12.1002256175434));
#117231=CARTESIAN_POINT('Ctrl Pts',(21.6704521373819,9.04350737951443,-12.1966331433727));
#117232=CARTESIAN_POINT('Ctrl Pts',(21.5541064924736,6.7363305172835,-11.0831182499555));
#117233=CARTESIAN_POINT('Ctrl Pts',(21.4377608475655,5.21954344324481,-9.0187039421408));
#117234=CARTESIAN_POINT('Ctrl Pts',(21.3214152026572,4.84535809285406,-6.48460381961909));
#117235=CARTESIAN_POINT('Ctrl Pts',(21.2050695577491,5.702915485133,-4.06976362634162));
#117236=CARTESIAN_POINT('Ctrl Pts',(21.0887239128409,7.58832332776442,-2.33877399674752));
#117237=CARTESIAN_POINT('Ctrl Pts',(20.9723782679327,10.071393582989,-1.68985471831868));
#117238=CARTESIAN_POINT('Ctrl Pts',(20.8560326230245,12.5555012697233,-2.28420337620227));
#117239=CARTESIAN_POINT('Ctrl Pts',(20.7009050964802,15.1484711142166,-4.52264463641619));
#117240=CARTESIAN_POINT('Ctrl Pts',(20.5069956882999,15.7229262950689,-9.1400595208437));
#117241=CARTESIAN_POINT('Ctrl Pts',(20.2743043984835,11.4791149812055,-12.8347932160127));
#117242=CARTESIAN_POINT('Ctrl Pts',(20.0803949903032,6.98475583574678,-11.6301128262941));
#117243=CARTESIAN_POINT('Ctrl Pts',(19.9252674637589,5.12461279872623,-8.75366018950281));
#117244=CARTESIAN_POINT('Ctrl Pts',(19.8089218188507,4.87791935403154,-6.21138096196604));
#117245=CARTESIAN_POINT('Ctrl Pts',(19.6925761739425,5.8625122183247,-3.84129425176305));
#117246=CARTESIAN_POINT('Ctrl Pts',(19.5762305290343,7.83658937295929,-2.21215115848727));
#117247=CARTESIAN_POINT('Ctrl Pts',(19.4598848841261,10.3464975445664,-1.69521904474282));
#117248=CARTESIAN_POINT('Ctrl Pts',(19.3435392392179,12.8049517620754,-2.41471954357795));
#117249=CARTESIAN_POINT('Ctrl Pts',(19.2271935943097,14.6408867640296,-4.20127828341279));
#117250=CARTESIAN_POINT('Ctrl Pts',(19.1108479494016,15.426161448925,-6.63978687694656));
#117251=CARTESIAN_POINT('Ctrl Pts',(18.9945023044933,14.9782424407922,-9.16203278420036));
#117252=CARTESIAN_POINT('Ctrl Pts',(18.8781566595852,13.4012753699925,-11.1809277310132));
#117253=CARTESIAN_POINT('Ctrl Pts',(18.761811014677,11.0625186928061,-12.2262884555702));
#117254=CARTESIAN_POINT('Ctrl Pts',(18.6454653697688,8.50650341460799,-12.0547549625971));
#117255=CARTESIAN_POINT('Ctrl Pts',(18.5291197248606,6.32839797170798,-10.7062461100025));
#117256=CARTESIAN_POINT('Ctrl Pts',(18.4127740799524,5.03535348126381,-8.49476372842595));
#117257=CARTESIAN_POINT('Ctrl Pts',(18.2964284350442,4.92844999693276,-5.93523409438871));
#117258=CARTESIAN_POINT('Ctrl Pts',(18.180082790136,6.03257984190088,-3.62362758376954));
#117259=CARTESIAN_POINT('Ctrl Pts',(18.0637371452278,8.09064926616096,-2.09819195226243));
#117260=CARTESIAN_POINT('Ctrl Pts',(17.9473915003196,10.6234591356293,-1.71410427383802));
#117261=CARTESIAN_POINT('Ctrl Pts',(17.8310458554114,13.0412395447846,-2.56082128275623));
#117262=CARTESIAN_POINT('Ctrl Pts',(17.7147002105032,14.7810690563125,-4.44113887229518));
#117263=CARTESIAN_POINT('Ctrl Pts',(17.598354565595,15.4377473099555,-6.91734398378451));
#117264=CARTESIAN_POINT('Ctrl Pts',(17.4820089206868,14.8585629802715,-9.41264012447143));
#117265=CARTESIAN_POINT('Ctrl Pts',(17.365659393706,13.177914321498,-11.3465348850005));
#117266=CARTESIAN_POINT('Ctrl Pts',(17.2880917483612,11.5845996678674,-11.9603779011799));
#117267=CARTESIAN_POINT('Ctrl Pts',(17.2493059846525,10.7620144760327,-12.0631388925593));
#117268=CARTESIAN_POINT('Ctrl Pts',(23.6939479204724,14.7863542679684,-8.25101022431757));
#117269=CARTESIAN_POINT('Ctrl Pts',(23.6551660388364,14.5831287004702,-9.00751231596158));
#117270=CARTESIAN_POINT('Ctrl Pts',(23.5776022755642,13.8012718976441,-10.4189287174808));
#117271=CARTESIAN_POINT('Ctrl Pts',(23.4612566306561,11.7725125602348,-11.740400440692));
#117272=CARTESIAN_POINT('Ctrl Pts',(23.3449109857478,9.36150678970984,-11.9578810059372));
#117273=CARTESIAN_POINT('Ctrl Pts',(23.2285653408397,7.12916157645969,-11.0210511445653));
#117274=CARTESIAN_POINT('Ctrl Pts',(23.1122196959314,5.59550259128015,-9.14789563612996));
#117275=CARTESIAN_POINT('Ctrl Pts',(22.9958740510233,5.11752049727005,-6.77463914492913));
#117276=CARTESIAN_POINT('Ctrl Pts',(22.879528406115,5.80656417108524,-4.45384546294059));
#117277=CARTESIAN_POINT('Ctrl Pts',(22.7631827612069,7.5021686101377,-2.72591334671949));
#117278=CARTESIAN_POINT('Ctrl Pts',(22.6468371162987,9.80953452025079,-1.99317356870946));
#117279=CARTESIAN_POINT('Ctrl Pts',(22.5304914713905,12.1914013165442,-2.42624316402794));
#117280=CARTESIAN_POINT('Ctrl Pts',(22.4141458264823,14.0931663649717,-3.92428411534862));
#117281=CARTESIAN_POINT('Ctrl Pts',(22.2978001815741,15.0720192602376,-6.138484863732));
#117282=CARTESIAN_POINT('Ctrl Pts',(22.1814545366659,14.9000299624285,-8.55328797261369));
#117283=CARTESIAN_POINT('Ctrl Pts',(22.0651088917577,13.6172674784149,-10.6064092325833));
#117284=CARTESIAN_POINT('Ctrl Pts',(21.9487632468495,11.5223678376368,-11.8198179451847));
#117285=CARTESIAN_POINT('Ctrl Pts',(21.8324176019413,9.10321467204312,-11.9109250368877));
#117286=CARTESIAN_POINT('Ctrl Pts',(21.7160719570331,6.92288515778683,-10.8586305958217));
#117287=CARTESIAN_POINT('Ctrl Pts',(21.5997263121249,5.48949022456477,-8.90771668078325));
#117288=CARTESIAN_POINT('Ctrl Pts',(21.4833806672167,5.13587738429453,-6.5129400255285));
#117289=CARTESIAN_POINT('Ctrl Pts',(21.3670350223085,5.94628673052317,-4.23086645249341));
#117290=CARTESIAN_POINT('Ctrl Pts',(21.2506893774004,7.72803585994387,-2.59504570547613));
#117291=CARTESIAN_POINT('Ctrl Pts',(21.1343437324921,10.0745882426698,-1.98180366136159));
#117292=CARTESIAN_POINT('Ctrl Pts',(21.017998087584,12.4221210194767,-2.54347534841603));
#117293=CARTESIAN_POINT('Ctrl Pts',(20.8628705610397,14.8725307709244,-4.65884830723382));
#117294=CARTESIAN_POINT('Ctrl Pts',(20.6689611528594,15.4154027136581,-9.02240019477693));
#117295=CARTESIAN_POINT('Ctrl Pts',(20.436269863043,11.4049138725019,-12.5139994105841));
#117296=CARTESIAN_POINT('Ctrl Pts',(20.2423604548627,7.15765218531772,-11.3755517033679));
#117297=CARTESIAN_POINT('Ctrl Pts',(20.0872329283184,5.39977881602929,-8.65724489168638));
#117298=CARTESIAN_POINT('Ctrl Pts',(19.9708872834102,5.16664844477492,-6.25473881422892));
#117299=CARTESIAN_POINT('Ctrl Pts',(19.854541638502,6.09710892081693,-4.01495820174247));
#117300=CARTESIAN_POINT('Ctrl Pts',(19.7381959935938,7.96265237096534,-2.47538452303399));
#117301=CARTESIAN_POINT('Ctrl Pts',(19.6218503486856,10.3345671358076,-1.98687305999249));
#117302=CARTESIAN_POINT('Ctrl Pts',(19.5055047037774,12.6578568573851,-2.66681580682442));
#117303=CARTESIAN_POINT('Ctrl Pts',(19.3891590588692,14.3928531364073,-4.3551505041687));
#117304=CARTESIAN_POINT('Ctrl Pts',(19.272813413961,15.1349538397841,-6.65959120149271));
#117305=CARTESIAN_POINT('Ctrl Pts',(19.1564677690528,14.7116611787767,-9.04316537988491));
#117306=CARTESIAN_POINT('Ctrl Pts',(19.0401221241446,13.2213949127782,-10.9510625640058));
#117307=CARTESIAN_POINT('Ctrl Pts',(18.9237764792364,11.0112218248761,-11.9389499159064));
#117308=CARTESIAN_POINT('Ctrl Pts',(18.8074308343282,8.59573489746441,-11.7768472424898));
#117309=CARTESIAN_POINT('Ctrl Pts',(18.69108518942,6.53738052504534,-10.5024786842401));
#117310=CARTESIAN_POINT('Ctrl Pts',(18.5747395445119,5.31542692802643,-8.41258241935363));
#117311=CARTESIAN_POINT('Ctrl Pts',(18.4583938996037,5.21440093999774,-5.99377435350435));
#117312=CARTESIAN_POINT('Ctrl Pts',(18.3420482546954,6.25782631755088,-3.80925873055534));
#117313=CARTESIAN_POINT('Ctrl Pts',(18.2257026097873,8.20274418733385,-2.36769073292162));
#117314=CARTESIAN_POINT('Ctrl Pts',(18.1093569648791,10.5963015269569,-2.0047199893085));
#117315=CARTESIAN_POINT('Ctrl Pts',(17.9930113199709,12.8811536643759,-2.8048849506466));
#117316=CARTESIAN_POINT('Ctrl Pts',(17.8766656750627,14.5253282813535,-4.58182368636311));
#117317=CARTESIAN_POINT('Ctrl Pts',(17.7603200301545,15.1459027163813,-6.92188836727878));
#117318=CARTESIAN_POINT('Ctrl Pts',(17.6439743852463,14.5985616308853,-9.27999446283346));
#117319=CARTESIAN_POINT('Ctrl Pts',(17.5276248582655,13.0103141350797,-11.1075647253793));
#117320=CARTESIAN_POINT('Ctrl Pts',(17.4500572129207,11.5045990675973,-11.6876589813532));
#117321=CARTESIAN_POINT('Ctrl Pts',(17.411271449212,10.7272391689664,-11.7847702284737));
#117322=CARTESIAN_POINT('Ctrl Pts',(23.8559133850319,14.5154275066996,-8.17822887259699));
#117323=CARTESIAN_POINT('Ctrl Pts',(23.8171315033958,14.324025209083,-8.89071913784739));
#117324=CARTESIAN_POINT('Ctrl Pts',(23.7395677401237,13.5876553206365,-10.2200220669534));
#117325=CARTESIAN_POINT('Ctrl Pts',(23.6232220952155,11.6769252718951,-11.4646131249179));
#117326=CARTESIAN_POINT('Ctrl Pts',(23.5068764503073,9.40618714712869,-11.6694410921238));
#117327=CARTESIAN_POINT('Ctrl Pts',(23.3905308053991,7.30371545446943,-10.7871141775044));
#117328=CARTESIAN_POINT('Ctrl Pts',(23.2741851604909,5.85928177844407,-9.02293522836227));
#117329=CARTESIAN_POINT('Ctrl Pts',(23.1578395155828,5.40910775684145,-6.78775020296697));
#117330=CARTESIAN_POINT('Ctrl Pts',(23.0414938706745,6.05806420434945,-4.60197580216125));
#117331=CARTESIAN_POINT('Ctrl Pts',(22.9251482257664,7.65502166141984,-2.97457142956318));
#117332=CARTESIAN_POINT('Ctrl Pts',(22.8088025808582,9.82814949210905,-2.28446103256568));
#117333=CARTESIAN_POINT('Ctrl Pts',(22.69245693595,12.0714438917243,-2.69233547765782));
#117334=CARTESIAN_POINT('Ctrl Pts',(22.5761112910418,13.8625679332368,-4.10322330804428));
#117335=CARTESIAN_POINT('Ctrl Pts',(22.4597656461336,14.7844730630341,-6.188606145658));
#117336=CARTESIAN_POINT('Ctrl Pts',(22.3434200012254,14.6224897694389,-8.46292068699072));
#117337=CARTESIAN_POINT('Ctrl Pts',(22.2270743563172,13.4143559221128,-10.3965953288256));
#117338=CARTESIAN_POINT('Ctrl Pts',(22.110728711409,11.4413334847428,-11.5394102728262));
#117339=CARTESIAN_POINT('Ctrl Pts',(21.9943830665008,9.1629219645718,-11.6252169304027));
#117340=CARTESIAN_POINT('Ctrl Pts',(21.8780374215926,7.10943979829016,-10.6341429416881));
#117341=CARTESIAN_POINT('Ctrl Pts',(21.7616917766844,5.75943700588474,-8.79672941942568));
#117342=CARTESIAN_POINT('Ctrl Pts',(21.6453461317762,5.42639667573499,-6.5412762314379));
#117343=CARTESIAN_POINT('Ctrl Pts',(21.529000486868,6.18965797591334,-4.39196927864519));
#117344=CARTESIAN_POINT('Ctrl Pts',(21.4126548419598,7.86774839212332,-2.85131741420474));
#117345=CARTESIAN_POINT('Ctrl Pts',(21.2963091970516,10.0777829023506,-2.2737526044045));
#117346=CARTESIAN_POINT('Ctrl Pts',(21.1799635521434,12.2887407692301,-2.80274732062977));
#117347=CARTESIAN_POINT('Ctrl Pts',(21.0248360255992,14.5965904276323,-4.79505197805147));
#117348=CARTESIAN_POINT('Ctrl Pts',(20.8309266174188,15.1078791322475,-8.90474086871017));
#117349=CARTESIAN_POINT('Ctrl Pts',(20.5982353276024,11.3307127637984,-12.1932056051556));
#117350=CARTESIAN_POINT('Ctrl Pts',(20.4043259194221,7.33054853488867,-11.1209905804417));
#117351=CARTESIAN_POINT('Ctrl Pts',(20.2491983928779,5.67494483333233,-8.56082959386996));
#117352=CARTESIAN_POINT('Ctrl Pts',(20.1328527479697,5.45537753551829,-6.29809666649179));
#117353=CARTESIAN_POINT('Ctrl Pts',(20.0165071030615,6.33170562330916,-4.18862215172188));
#117354=CARTESIAN_POINT('Ctrl Pts',(19.9001614581533,8.08871536897138,-2.73861788758071));
#117355=CARTESIAN_POINT('Ctrl Pts',(19.7838158132451,10.3226367270489,-2.27852707524217));
#117356=CARTESIAN_POINT('Ctrl Pts',(19.6674701683369,12.510761952695,-2.91891207007088));
#117357=CARTESIAN_POINT('Ctrl Pts',(19.5511245234287,14.1448195087852,-4.50902272492462));
#117358=CARTESIAN_POINT('Ctrl Pts',(19.4347788785205,14.843746230643,-6.67939552603887));
#117359=CARTESIAN_POINT('Ctrl Pts',(19.3184332336123,14.4450799167611,-8.92429797556946));
#117360=CARTESIAN_POINT('Ctrl Pts',(19.2020875887041,13.0415144555639,-10.7211973969982));
#117361=CARTESIAN_POINT('Ctrl Pts',(19.0857419437959,10.959924956946,-11.6516113762426));
#117362=CARTESIAN_POINT('Ctrl Pts',(18.9693962988877,8.68496638032083,-11.4989395223824));
#117363=CARTESIAN_POINT('Ctrl Pts',(18.8530506539795,6.7463630783827,-10.2987112584779));
#117364=CARTESIAN_POINT('Ctrl Pts',(18.7367050090713,5.59550037478904,-8.33040111028128));
#117365=CARTESIAN_POINT('Ctrl Pts',(18.6203593641631,5.50035188306271,-6.05231461262));
#117366=CARTESIAN_POINT('Ctrl Pts',(18.5040137192549,6.48307279320089,-3.99488987734113));
#117367=CARTESIAN_POINT('Ctrl Pts',(18.3876680743467,8.31483910850671,-2.63718951358079));
#117368=CARTESIAN_POINT('Ctrl Pts',(18.2713224294385,10.5691439182845,-2.29533570477897));
#117369=CARTESIAN_POINT('Ctrl Pts',(18.1549767845304,12.7210677839672,-3.04894861853697));
#117370=CARTESIAN_POINT('Ctrl Pts',(18.0386311396222,14.2695875063947,-4.72250850043103));
#117371=CARTESIAN_POINT('Ctrl Pts',(17.922285494714,14.8540581228072,-6.92643275077305));
#117372=CARTESIAN_POINT('Ctrl Pts',(17.8059398498058,14.3385602814992,-9.14734880119549));
#117373=CARTESIAN_POINT('Ctrl Pts',(17.6895903228249,12.8427139486614,-10.8685945657582));
#117374=CARTESIAN_POINT('Ctrl Pts',(17.6120226774801,11.4245984673272,-11.4149400615265));
#117375=CARTESIAN_POINT('Ctrl Pts',(17.5732369137714,10.6924638619,-11.5064015643881));
#117376=CARTESIAN_POINT('Ctrl Pts',(24.0178788495913,14.2445007454307,-8.1054475208764));
#117377=CARTESIAN_POINT('Ctrl Pts',(23.9790969679552,14.0649217176957,-8.77392595973318));
#117378=CARTESIAN_POINT('Ctrl Pts',(23.9015332046831,13.374038743629,-10.0211154164259));
#117379=CARTESIAN_POINT('Ctrl Pts',(23.7851875597749,11.5813379835554,-11.1888258091439));
#117380=CARTESIAN_POINT('Ctrl Pts',(23.6688419148667,9.45086750454755,-11.3810011783102));
#117381=CARTESIAN_POINT('Ctrl Pts',(23.5524962699585,7.47826933247917,-10.5531772104435));
#117382=CARTESIAN_POINT('Ctrl Pts',(23.4361506250503,6.123060965608,-8.89797482059457));
#117383=CARTESIAN_POINT('Ctrl Pts',(23.3198049801421,5.70069501641282,-6.80086126100482));
#117384=CARTESIAN_POINT('Ctrl Pts',(23.2034593352339,6.30956423761369,-4.75010614138192));
#117385=CARTESIAN_POINT('Ctrl Pts',(23.0871136903257,7.80787471270198,-3.22322951240687));
#117386=CARTESIAN_POINT('Ctrl Pts',(22.9707680454175,9.84676446396732,-2.5757484964219));
#117387=CARTESIAN_POINT('Ctrl Pts',(22.8544224005093,11.9514864669044,-2.95842779128772));
#117388=CARTESIAN_POINT('Ctrl Pts',(22.7380767556011,13.6319695015019,-4.28216250073993));
#117389=CARTESIAN_POINT('Ctrl Pts',(22.6217311106929,14.4969268658308,-6.238727427584));
#117390=CARTESIAN_POINT('Ctrl Pts',(22.5053854657848,14.3449495764493,-8.37255340136776));
#117391=CARTESIAN_POINT('Ctrl Pts',(22.3890398208766,13.2114443658107,-10.1867814250677));
#117392=CARTESIAN_POINT('Ctrl Pts',(22.2726941759684,11.3602991318489,-11.2590026004677));
#117393=CARTESIAN_POINT('Ctrl Pts',(22.1563485310602,9.22262925710048,-11.3395088239177));
#117394=CARTESIAN_POINT('Ctrl Pts',(22.040002886152,7.29599443879349,-10.4096552875544));
#117395=CARTESIAN_POINT('Ctrl Pts',(21.9236572412438,6.02938378720469,-8.68574215806813));
#117396=CARTESIAN_POINT('Ctrl Pts',(21.8073115963356,5.71691596717546,-6.56961243734728));
#117397=CARTESIAN_POINT('Ctrl Pts',(21.6909659514274,6.43302922130351,-4.55307210479699));
#117398=CARTESIAN_POINT('Ctrl Pts',(21.5746203065192,8.00746092430277,-3.10758912293336));
#117399=CARTESIAN_POINT('Ctrl Pts',(21.458274661611,10.0809775620313,-2.56570154744741));
#117400=CARTESIAN_POINT('Ctrl Pts',(21.3419290167028,12.1553605189835,-3.06201929284352));
#117401=CARTESIAN_POINT('Ctrl Pts',(21.1868014901586,14.3206500843401,-4.93125564886911));
#117402=CARTESIAN_POINT('Ctrl Pts',(20.9928920819782,14.8003555508367,-8.7870815426434));
#117403=CARTESIAN_POINT('Ctrl Pts',(20.7602007921619,11.2565116550948,-11.8724117997271));
#117404=CARTESIAN_POINT('Ctrl Pts',(20.5662913839815,7.50344488445961,-10.8664294575155));
#117405=CARTESIAN_POINT('Ctrl Pts',(20.4111638574373,5.95011085063539,-8.46441429605354));
#117406=CARTESIAN_POINT('Ctrl Pts',(20.294818212529,5.74410662626167,-6.34145451875465));
#117407=CARTESIAN_POINT('Ctrl Pts',(20.1784725676209,6.56630232580139,-4.36228610170129));
#117408=CARTESIAN_POINT('Ctrl Pts',(20.0621269227127,8.21477836697742,-3.00185125212742));
#117409=CARTESIAN_POINT('Ctrl Pts',(19.9457812778045,10.31070631829,-2.57018109049185));
#117410=CARTESIAN_POINT('Ctrl Pts',(19.8294356328963,12.3636670480047,-3.17100833331735));
#117411=CARTESIAN_POINT('Ctrl Pts',(19.7130899879881,13.896785881163,-4.66289494568054));
#117412=CARTESIAN_POINT('Ctrl Pts',(19.5967443430799,14.5525386215021,-6.69919985058501));
#117413=CARTESIAN_POINT('Ctrl Pts',(19.4803986981717,14.1784986547455,-8.80543057125401));
#117414=CARTESIAN_POINT('Ctrl Pts',(19.3640530532635,12.8616339983496,-10.4913322299906));
#117415=CARTESIAN_POINT('Ctrl Pts',(19.2477074083553,10.9086280890158,-11.3642728365788));
#117416=CARTESIAN_POINT('Ctrl Pts',(19.1313617634471,8.77419786317726,-11.221031802275));
#117417=CARTESIAN_POINT('Ctrl Pts',(19.0150161185389,6.95534563172006,-10.0949438327155));
#117418=CARTESIAN_POINT('Ctrl Pts',(18.8986704736307,5.87557382155166,-8.24821980120896));
#117419=CARTESIAN_POINT('Ctrl Pts',(18.7823248287225,5.78630282612769,-6.11085487173564));
#117420=CARTESIAN_POINT('Ctrl Pts',(18.6659791838143,6.70831926885089,-4.18052102412694));
#117421=CARTESIAN_POINT('Ctrl Pts',(18.5496335389061,8.42693402967958,-2.90668829423997));
#117422=CARTESIAN_POINT('Ctrl Pts',(18.4332878939979,10.5419863096122,-2.58595142024945));
#117423=CARTESIAN_POINT('Ctrl Pts',(18.3169422490897,12.5609819035585,-3.29301228642734));
#117424=CARTESIAN_POINT('Ctrl Pts',(18.2005966041815,14.0138467314357,-4.86319331449896));
#117425=CARTESIAN_POINT('Ctrl Pts',(18.0842509592733,14.5622135292331,-6.93097713426731));
#117426=CARTESIAN_POINT('Ctrl Pts',(17.9679053143652,14.078558932113,-9.01470313955753));
#117427=CARTESIAN_POINT('Ctrl Pts',(17.8515557873843,12.6751137622431,-10.629624406137));
#117428=CARTESIAN_POINT('Ctrl Pts',(17.7739881420395,11.3445978670571,-11.1422211416999));
#117429=CARTESIAN_POINT('Ctrl Pts',(17.7352023783309,10.6576885548338,-11.2280329003024));
#117430=CARTESIAN_POINT('Ctrl Pts',(17.734,10.6581555755053,-11.2300936493755));
#117431=CARTESIAN_POINT('Ctrl Pts',(17.734,10.7871580301293,-11.2265276116833));
#117432=CARTESIAN_POINT('Ctrl Pts',(17.734,10.9158060854873,-11.2169788999138));
#117433=CARTESIAN_POINT('Ctrl Pts',(17.734,11.0437268225087,-11.2016549886172));
#117434=CARTESIAN_POINT('Ctrl Pts',(17.734,11.1739880982412,-11.1860506989516));
#117435=CARTESIAN_POINT('Ctrl Pts',(17.7339999999999,11.3034959147556,-11.1644579899712));
#117436=CARTESIAN_POINT('Ctrl Pts',(17.734,11.4318673763278,-11.1370431572385));
#117437=CARTESIAN_POINT('Ctrl Pts',(17.734,11.4884530911241,-11.1249587898316));
#117438=CARTESIAN_POINT('Ctrl Pts',(17.734,11.5448180845801,-11.1117424890276));
#117439=CARTESIAN_POINT('Ctrl Pts',(17.734,11.6009296449061,-11.0974052968746));
#117440=CARTESIAN_POINT('Ctrl Pts',(17.7339999999999,11.6231422455803,-11.0917297048534));
#117441=CARTESIAN_POINT('Ctrl Pts',(17.734,11.6453151296432,-11.0858784376901));
#117442=CARTESIAN_POINT('Ctrl Pts',(17.734,11.6674462597462,-11.0798520970063));
#117443=CARTESIAN_POINT('Ctrl Pts',(17.734,11.6909691969026,-11.0734467651264));
#117444=CARTESIAN_POINT('Ctrl Pts',(17.7339999999999,11.7144371000566,-11.0668457533736));
#117445=CARTESIAN_POINT('Ctrl Pts',(17.7339999999999,11.7378417469922,-11.0600519299264));
#117446=CARTESIAN_POINT('Ctrl Pts',(17.7339999999999,11.8666178352729,-11.0226712332466));
#117447=CARTESIAN_POINT('Ctrl Pts',(17.734,11.9935344010332,-10.9794425381218));
#117448=CARTESIAN_POINT('Ctrl Pts',(17.734,12.1181943387372,-10.9305490461558));
#117449=CARTESIAN_POINT('Ctrl Pts',(17.734,12.2170317257716,-10.8917835447612));
#117450=CARTESIAN_POINT('Ctrl Pts',(17.7339999999999,12.3144508717194,-10.8494559613376));
#117451=CARTESIAN_POINT('Ctrl Pts',(17.734,12.4102527649422,-10.8036343689628));
#117452=CARTESIAN_POINT('Ctrl Pts',(17.734,12.4582931021382,-10.7806569029182));
#117453=CARTESIAN_POINT('Ctrl Pts',(17.7339999999999,12.5059267258685,-10.7568005259236));
#117454=CARTESIAN_POINT('Ctrl Pts',(17.7339999999999,12.5531281105939,-10.7320719318602));
#117455=CARTESIAN_POINT('Ctrl Pts',(17.7339999999999,12.5796828219838,-10.7181600374899));
#117456=CARTESIAN_POINT('Ctrl Pts',(17.734,12.6061007231861,-10.703972063894));
#117457=CARTESIAN_POINT('Ctrl Pts',(17.734,12.6323772088884,-10.6895090305751));
#117458=CARTESIAN_POINT('Ctrl Pts',(17.734,12.6494661520011,-10.6801029799934));
#117459=CARTESIAN_POINT('Ctrl Pts',(17.734,12.6664940896698,-10.6705811847365));
#117460=CARTESIAN_POINT('Ctrl Pts',(17.734,12.683449666574,-10.6609498639215));
#117461=CARTESIAN_POINT('Ctrl Pts',(17.734,12.6867649951574,-10.6590666491319));
#117462=CARTESIAN_POINT('Ctrl Pts',(17.7339999999999,12.6900776631735,-10.6571791889994));
#117463=CARTESIAN_POINT('Ctrl Pts',(17.7339999999999,12.6933876620448,-10.6552874881657));
#117464=CARTESIAN_POINT('Ctrl Pts',(17.734,12.813721983353,-10.5865150973585));
#117465=CARTESIAN_POINT('Ctrl Pts',(17.7339999999999,12.9305291947834,-10.5121431425042));
#117466=CARTESIAN_POINT('Ctrl Pts',(17.7339999999999,13.0435566004255,-10.4326032510522));
#117467=CARTESIAN_POINT('Ctrl Pts',(17.7339999999999,13.1542860408063,-10.3546804887062));
#117468=CARTESIAN_POINT('Ctrl Pts',(17.734,13.2613883832878,-10.2717971251544));
#117469=CARTESIAN_POINT('Ctrl Pts',(17.734,13.3646136018083,-10.1843046204669));
#117470=CARTESIAN_POINT('Ctrl Pts',(17.734,13.4710521658324,-10.0940885211912));
#117471=CARTESIAN_POINT('Ctrl Pts',(17.734,13.5733692644385,-9.99897159633853));
#117472=CARTESIAN_POINT('Ctrl Pts',(17.734,13.6712668291686,-9.89928713892356));
#117473=CARTESIAN_POINT('Ctrl Pts',(17.734,13.7691643938987,-9.79960268150859));
#117474=CARTESIAN_POINT('Ctrl Pts',(17.734,13.8626431607924,-9.69535014068121));
#117475=CARTESIAN_POINT('Ctrl Pts',(17.734,13.9513699801085,-9.58681812087919));
#117476=CARTESIAN_POINT('Ctrl Pts',(17.734,13.9628634835586,-9.57275908941993));
#117477=CARTESIAN_POINT('Ctrl Pts',(17.734,13.9742785921472,-9.55862643429634));
#117478=CARTESIAN_POINT('Ctrl Pts',(17.734,13.9856099775934,-9.5444264491211));
#117479=CARTESIAN_POINT('Ctrl Pts',(17.734,14.0729113490609,-9.43502427702995));
#117480=CARTESIAN_POINT('Ctrl Pts',(17.734,14.155041858068,-9.32188662452608));
#117481=CARTESIAN_POINT('Ctrl Pts',(17.734,14.2317472591746,-9.20538350790436));
#117482=CARTESIAN_POINT('Ctrl Pts',(17.734,14.2502066068323,-9.17734673993373));
#117483=CARTESIAN_POINT('Ctrl Pts',(17.734,14.2683516627921,-9.14911485201464));
#117484=CARTESIAN_POINT('Ctrl Pts',(17.734,14.2861786693898,-9.12069260839312));
#117485=CARTESIAN_POINT('Ctrl Pts',(17.734,14.3596274174382,-9.00359060367398));
#117486=CARTESIAN_POINT('Ctrl Pts',(17.734,14.4276801174427,-8.88326038142567));
#117487=CARTESIAN_POINT('Ctrl Pts',(17.734,14.4902884333848,-8.76012784854764));
#117488=CARTESIAN_POINT('Ctrl Pts',(17.734,14.5537529998899,-8.63531131732177));
#117489=CARTESIAN_POINT('Ctrl Pts',(17.734,14.6116236543302,-8.50761468832594));
#117490=CARTESIAN_POINT('Ctrl Pts',(17.734,14.6638094340167,-8.37744644945232));
#117491=CARTESIAN_POINT('Ctrl Pts',(17.734,14.7100740696579,-8.26204746184093));
#117492=CARTESIAN_POINT('Ctrl Pts',(17.734,14.7518702709579,-8.14470509092101));
#117493=CARTESIAN_POINT('Ctrl Pts',(17.734,14.7891046475072,-8.02568745899151));
#117494=CARTESIAN_POINT('Ctrl Pts',(17.734,14.7957588699923,-8.0044176036614));
#117495=CARTESIAN_POINT('Ctrl Pts',(17.734,14.802267320164,-7.98309421356168));
#117496=CARTESIAN_POINT('Ctrl Pts',(17.734,14.8086293625773,-7.9617187827321));
#117497=CARTESIAN_POINT('Ctrl Pts',(17.734,14.8141582507119,-7.94314261517331));
#117498=CARTESIAN_POINT('Ctrl Pts',(17.734,14.8195767038318,-7.92452645243315));
#117499=CARTESIAN_POINT('Ctrl Pts',(17.734,14.8248800133524,-7.90588690657763));
#117500=CARTESIAN_POINT('Ctrl Pts',(17.734,14.8642211214105,-7.76761468527757));
#117501=CARTESIAN_POINT('Ctrl Pts',(17.734,14.8972903477015,-7.62785672464364));
#117502=CARTESIAN_POINT('Ctrl Pts',(17.734,14.9240435546541,-7.48706785777855));
#117503=CARTESIAN_POINT('Ctrl Pts',(17.734,14.9507706801502,-7.34641624469049));
#117504=CARTESIAN_POINT('Ctrl Pts',(17.734,14.9711943919531,-7.20473499473391));
#117505=CARTESIAN_POINT('Ctrl Pts',(17.734,14.9852278277044,-7.06244825044858));
#117506=CARTESIAN_POINT('Ctrl Pts',(17.734,14.9897675457622,-7.01641948644057));
#117507=CARTESIAN_POINT('Ctrl Pts',(17.734,14.9936381823968,-6.9703271759923));
#117508=CARTESIAN_POINT('Ctrl Pts',(17.734,14.9968357553433,-6.92418521713769));
#117509=CARTESIAN_POINT('Ctrl Pts',(17.7339999999999,15.0067323514289,-6.78137429866482));
#117510=CARTESIAN_POINT('Ctrl Pts',(17.734,15.010185425558,-6.63808849971123));
#117511=CARTESIAN_POINT('Ctrl Pts',(17.734,15.0073112040798,-6.49472810706362));
#117512=CARTESIAN_POINT('Ctrl Pts',(17.734,15.0056440306924,-6.41157284806938));
#117513=CARTESIAN_POINT('Ctrl Pts',(17.734,15.0018470671246,-6.32839227527476));
#117514=CARTESIAN_POINT('Ctrl Pts',(17.734,14.9959350165701,-6.24526375434569));
#117515=CARTESIAN_POINT('Ctrl Pts',(17.734,14.9930494071184,-6.20468960101485));
#117516=CARTESIAN_POINT('Ctrl Pts',(17.734,14.9896598294849,-6.16412784684823));
#117517=CARTESIAN_POINT('Ctrl Pts',(17.734,14.9857674896188,-6.12358750933691));
#117518=CARTESIAN_POINT('Ctrl Pts',(17.734,14.9839181537182,-6.10432590727623));
#117519=CARTESIAN_POINT('Ctrl Pts',(17.734,14.9819550242892,-6.08506643814876));
#117520=CARTESIAN_POINT('Ctrl Pts',(17.734,14.9798791802301,-6.06581902520355));
#117521=CARTESIAN_POINT('Ctrl Pts',(17.734,14.9642028796882,-5.92046695568585));
#117522=CARTESIAN_POINT('Ctrl Pts',(17.734,14.9421349343852,-5.77608373015697));
#117523=CARTESIAN_POINT('Ctrl Pts',(17.734,14.9138625332143,-5.63308993321275));
#117524=CARTESIAN_POINT('Ctrl Pts',(17.734,14.8852999124013,-5.48862828752365));
#117525=CARTESIAN_POINT('Ctrl Pts',(17.734,14.8504048158092,-5.34558398961965));
#117526=CARTESIAN_POINT('Ctrl Pts',(17.734,14.809317815667,-5.20437943584449));
#117527=CARTESIAN_POINT('Ctrl Pts',(17.734,14.7681579286984,-5.06292439038676));
#117528=CARTESIAN_POINT('Ctrl Pts',(17.734,14.7207840951756,-4.92331482471784));
#117529=CARTESIAN_POINT('Ctrl Pts',(17.734,14.6672857084543,-4.78597583902191));
#117530=CARTESIAN_POINT('Ctrl Pts',(17.734,14.6372084702442,-4.70876271837517));
#117531=CARTESIAN_POINT('Ctrl Pts',(17.734,14.6051944642096,-4.63226735310747));
#117532=CARTESIAN_POINT('Ctrl Pts',(17.734,14.5712524834494,-4.55656680407633));
#117533=CARTESIAN_POINT('Ctrl Pts',(17.734,14.5209818578362,-4.44444859901506));
#117534=CARTESIAN_POINT('Ctrl Pts',(17.734,14.4664830452091,-4.33407329976893));
#117535=CARTESIAN_POINT('Ctrl Pts',(17.734,14.4079024230562,-4.22562346067728));
#117536=CARTESIAN_POINT('Ctrl Pts',(23.534,15.0539061944433,-8.32288496556903));
#117537=CARTESIAN_POINT('Ctrl Pts',(23.534,15.0045196831565,-8.46102105477097));
#117538=CARTESIAN_POINT('Ctrl Pts',(23.534,14.9491584466399,-8.59666359933272));
#117539=CARTESIAN_POINT('Ctrl Pts',(23.534,14.8880945730865,-8.72949016701654));
#117540=CARTESIAN_POINT('Ctrl Pts',(23.534,14.8263802252152,-8.86373165101629));
#117541=CARTESIAN_POINT('Ctrl Pts',(23.534,14.7588406646494,-8.9950975097176));
#117542=CARTESIAN_POINT('Ctrl Pts',(23.534,14.6857106710858,-9.12322928795019));
#117543=CARTESIAN_POINT('Ctrl Pts',(23.534,14.6128819085607,-9.25083327632891));
#117544=CARTESIAN_POINT('Ctrl Pts',(23.534,14.5345081505571,-9.37523035923853));
#117545=CARTESIAN_POINT('Ctrl Pts',(23.534,14.4507831744512,-9.49603193130466));
#117546=CARTESIAN_POINT('Ctrl Pts',(23.534,14.3684650046213,-9.61480370990148));
#117547=CARTESIAN_POINT('Ctrl Pts',(23.534,14.2809734005509,-9.73010024311516));
#117548=CARTESIAN_POINT('Ctrl Pts',(23.534,14.1884635407854,-9.84151116501367));
#117549=CARTESIAN_POINT('Ctrl Pts',(23.534,14.1636970862179,-9.87133775368768));
#117550=CARTESIAN_POINT('Ctrl Pts',(23.534,14.1385708227766,-9.90088559984928));
#117551=CARTESIAN_POINT('Ctrl Pts',(23.534,14.1130874412093,-9.9301462552455));
#117552=CARTESIAN_POINT('Ctrl Pts',(23.534,14.0994446628436,-9.94581123421829));
#117553=CARTESIAN_POINT('Ctrl Pts',(23.534,14.0856995289216,-9.96139389704753));
#117554=CARTESIAN_POINT('Ctrl Pts',(23.534,14.0718524398192,-9.97689291659844));
#117555=CARTESIAN_POINT('Ctrl Pts',(23.534,14.0595282691968,-9.99068733649516));
#117556=CARTESIAN_POINT('Ctrl Pts',(23.534,14.0471248899774,-10.0044136985475));
#117557=CARTESIAN_POINT('Ctrl Pts',(23.534,14.0346501013912,-10.0180631245397));
#117558=CARTESIAN_POINT('Ctrl Pts',(23.534,13.9325629744592,-10.129762867921));
#117559=CARTESIAN_POINT('Ctrl Pts',(23.534,13.8255589167938,-10.2364694610508));
#117560=CARTESIAN_POINT('Ctrl Pts',(23.534,13.7138822995671,-10.3377901011926));
#117561=CARTESIAN_POINT('Ctrl Pts',(23.534,13.6072656917372,-10.4345199558688));
#117562=CARTESIAN_POINT('Ctrl Pts',(23.534,13.4963893994937,-10.5263409917788));
#117563=CARTESIAN_POINT('Ctrl Pts',(23.534,13.3816361432654,-10.6130491512947));
#117564=CARTESIAN_POINT('Ctrl Pts',(23.534,13.2675216549448,-10.6992746544448));
#117565=CARTESIAN_POINT('Ctrl Pts',(23.534,13.1495724821822,-10.7804443135787));
#117566=CARTESIAN_POINT('Ctrl Pts',(23.534,13.028145213054,-10.8563104469597));
#117567=CARTESIAN_POINT('Ctrl Pts',(23.534,12.9228679009085,-10.9220863032608));
#117568=CARTESIAN_POINT('Ctrl Pts',(23.534,12.8149755625505,-10.9838749598991));
#117569=CARTESIAN_POINT('Ctrl Pts',(23.534,12.7046950051531,-11.0414837392859));
#117570=CARTESIAN_POINT('Ctrl Pts',(23.534,12.6704660549416,-11.0593643892202));
#117571=CARTESIAN_POINT('Ctrl Pts',(23.534,12.6360070180388,-11.0768421453942));
#117572=CARTESIAN_POINT('Ctrl Pts',(23.534,12.6013246618057,-11.0939106397649));
#117573=CARTESIAN_POINT('Ctrl Pts',(23.534,12.5775343548302,-11.1056187462719));
#117574=CARTESIAN_POINT('Ctrl Pts',(23.534,12.5536338344587,-11.1171366062184));
#117575=CARTESIAN_POINT('Ctrl Pts',(23.534,12.5296548188552,-11.1284484392924));
#117576=CARTESIAN_POINT('Ctrl Pts',(23.534,12.4026030627483,-11.1883836877031));
#117577=CARTESIAN_POINT('Ctrl Pts',(23.534,12.2732186532335,-11.2426060623178));
#117578=CARTESIAN_POINT('Ctrl Pts',(23.534,12.1418579788867,-11.2909272251374));
#117579=CARTESIAN_POINT('Ctrl Pts',(23.534,12.0110656904146,-11.3390393066126));
#117580=CARTESIAN_POINT('Ctrl Pts',(23.534,11.8783134757111,-11.381301368659));
#117581=CARTESIAN_POINT('Ctrl Pts',(23.534,11.7439408942886,-11.4174776418709));
#117582=CARTESIAN_POINT('Ctrl Pts',(23.534,11.7185306168275,-11.4243186888322));
#117583=CARTESIAN_POINT('Ctrl Pts',(23.534,11.6930623778329,-11.4309419582457));
#117584=CARTESIAN_POINT('Ctrl Pts',(23.534,11.6675384567621,-11.4373456433974));
#117585=CARTESIAN_POINT('Ctrl Pts',(23.534,11.5320041155766,-11.4713497936919));
#117586=CARTESIAN_POINT('Ctrl Pts',(23.534,11.394899148674,-11.4991663992332));
#117587=CARTESIAN_POINT('Ctrl Pts',(23.534,11.2566535581235,-11.5207487746459));
#117588=CARTESIAN_POINT('Ctrl Pts',(23.534,11.1395174117289,-11.5390356239828));
#117589=CARTESIAN_POINT('Ctrl Pts',(23.534,11.0215621487013,-11.5528458727715));
#117590=CARTESIAN_POINT('Ctrl Pts',(23.534,10.9030568789718,-11.5621227836795));
#117591=CARTESIAN_POINT('Ctrl Pts',(23.534,10.8727885717626,-11.5644922680911));
#117592=CARTESIAN_POINT('Ctrl Pts',(23.534,10.842484435087,-11.5665658756357));
#117593=CARTESIAN_POINT('Ctrl Pts',(23.534,10.8121490716819,-11.5683423926637));
#117594=CARTESIAN_POINT('Ctrl Pts',(23.534,10.7942046025595,-11.5693932670024));
#117595=CARTESIAN_POINT('Ctrl Pts',(23.5339999999999,10.7762590661863,-11.5703396029876));
#117596=CARTESIAN_POINT('Ctrl Pts',(23.5339999999999,10.7583140714215,-11.5711814532735));
#117597=CARTESIAN_POINT('Ctrl Pts',(23.534,10.621315610092,-11.5776084372518));
#117598=CARTESIAN_POINT('Ctrl Pts',(23.534,10.4843351016943,-11.5779507199327));
#117599=CARTESIAN_POINT('Ctrl Pts',(23.534,10.3477779769602,-11.5722201804618));
#117600=CARTESIAN_POINT('Ctrl Pts',(23.534,10.2117250436855,-11.566510799089));
#117601=CARTESIAN_POINT('Ctrl Pts',(23.5339999999999,10.0760915866747,-11.5547732226133));
#117602=CARTESIAN_POINT('Ctrl Pts',(23.534,9.94128731876771,-11.5369684475271));
#117603=CARTESIAN_POINT('Ctrl Pts',(23.534,9.80868446685906,-11.5194544326471));
#117604=CARTESIAN_POINT('Ctrl Pts',(23.5339999999999,9.67688326966917,-11.4960695457184));
#117605=CARTESIAN_POINT('Ctrl Pts',(23.534,9.54629292155958,-11.4667302088915));
#117606=CARTESIAN_POINT('Ctrl Pts',(23.534,9.5112464654664,-11.4588564280586));
#117607=CARTESIAN_POINT('Ctrl Pts',(23.534,9.47628735692625,-11.4505535423215));
#117608=CARTESIAN_POINT('Ctrl Pts',(23.534,9.44142384068047,-11.4418193834442));
#117609=CARTESIAN_POINT('Ctrl Pts',(23.534,9.35465567581842,-11.4200818475038));
#117610=CARTESIAN_POINT('Ctrl Pts',(23.534,9.26847914064438,-11.395673426388));
#117611=CARTESIAN_POINT('Ctrl Pts',(23.534,9.18301437324066,-11.3686311001959));
#117612=CARTESIAN_POINT('Ctrl Pts',(23.5339999999999,9.15095469784314,-11.3584869410757));
#117613=CARTESIAN_POINT('Ctrl Pts',(23.534,9.11899524917182,-11.347972079119));
#117614=CARTESIAN_POINT('Ctrl Pts',(23.534,9.08714263326125,-11.3370882239502));
#117615=CARTESIAN_POINT('Ctrl Pts',(23.534,9.06138445712602,-11.3282868037072));
#117616=CARTESIAN_POINT('Ctrl Pts',(23.534,9.03570611702107,-11.3192474074339));
#117617=CARTESIAN_POINT('Ctrl Pts',(23.534,9.01012249912345,-11.3099758408373));
#117618=CARTESIAN_POINT('Ctrl Pts',(23.534,8.8838168776646,-11.2642023702683));
#117619=CARTESIAN_POINT('Ctrl Pts',(23.534,8.75972821615212,-11.2127431096887));
#117620=CARTESIAN_POINT('Ctrl Pts',(23.534,8.63823633729656,-11.1557838964956));
#117621=CARTESIAN_POINT('Ctrl Pts',(23.534,8.51762503020503,-11.0992375230357));
#117622=CARTESIAN_POINT('Ctrl Pts',(23.534,8.39957237065447,-11.0372701273009));
#117623=CARTESIAN_POINT('Ctrl Pts',(23.534,8.28448331249122,-10.970024793541));
#117624=CARTESIAN_POINT('Ctrl Pts',(23.534,8.2674356587266,-10.9600640276305));
#117625=CARTESIAN_POINT('Ctrl Pts',(23.534,8.25045309991395,-10.9499873953753));
#117626=CARTESIAN_POINT('Ctrl Pts',(23.534,8.23353702790624,-10.939795299223));
#117627=CARTESIAN_POINT('Ctrl Pts',(23.534,8.20315452082413,-10.9214895463633));
#117628=CARTESIAN_POINT('Ctrl Pts',(23.534,8.17298647883074,-10.902811329405));
#117629=CARTESIAN_POINT('Ctrl Pts',(23.534,8.14304114129206,-10.8837628607093));
#117630=CARTESIAN_POINT('Ctrl Pts',(23.5339999999999,8.12583577094011,-10.8728183870288));
#117631=CARTESIAN_POINT('Ctrl Pts',(23.534,8.1087059434679,-10.8617529204478));
#117632=CARTESIAN_POINT('Ctrl Pts',(23.534,8.09166038518002,-10.8505717991687));
#117633=CARTESIAN_POINT('Ctrl Pts',(23.534,7.98236466033434,-10.778878708561));
#117634=CARTESIAN_POINT('Ctrl Pts',(23.534,7.87644328077352,-10.7023783007895));
#117635=CARTESIAN_POINT('Ctrl Pts',(23.5339999999999,7.77426954147455,-10.6212231772217));
#117636=CARTESIAN_POINT('Ctrl Pts',(23.5339999999999,7.70156836402741,-10.5634776833234));
#117637=CARTESIAN_POINT('Ctrl Pts',(23.534,7.63076526501317,-10.5033747155762));
#117638=CARTESIAN_POINT('Ctrl Pts',(23.534,7.56200744420826,-10.4409593356367));
#117639=CARTESIAN_POINT('Ctrl Pts',(23.534,7.48528237325109,-10.3713116301304));
#117640=CARTESIAN_POINT('Ctrl Pts',(23.534,7.41110370365363,-10.298784417752));
#117641=CARTESIAN_POINT('Ctrl Pts',(23.5339999999999,7.33961515870573,-10.2235362531339));
#117642=CARTESIAN_POINT('Ctrl Pts',(-17.1175857387455,20.5721719462546,
-0.00214206224876584));
#117643=CARTESIAN_POINT('Ctrl Pts',(-16.6641680440313,20.0337688721201,
-0.0445526553076215));
#117644=CARTESIAN_POINT('Ctrl Pts',(-16.3459143283547,18.477787514409,-0.129355183926955));
#117645=CARTESIAN_POINT('Ctrl Pts',(-18.0613963234494,16.802775720219,-0.256549648106768));
#117646=CARTESIAN_POINT('Ctrl Pts',(-20.3933471209293,17.343653714663,-0.383725454788201));
#117647=CARTESIAN_POINT('Ctrl Pts',(-21.203092243631,19.5945946034862,-0.510901261469636));
#117648=CARTESIAN_POINT('Ctrl Pts',(-19.7475288885744,21.4952120560344,
-0.638077068151069));
#117649=CARTESIAN_POINT('Ctrl Pts',(-17.3621513494713,21.2993774656764,
-0.765252874832505));
#117650=CARTESIAN_POINT('Ctrl Pts',(-16.2353413405934,19.188016346975,-0.892428681513937));
#117651=CARTESIAN_POINT('Ctrl Pts',(-17.4009051420832,17.0975180849442,
-1.01960448819538));
#117652=CARTESIAN_POINT('Ctrl Pts',(-19.7894957664261,16.9461241370553,
-1.14678029487681));
#117653=CARTESIAN_POINT('Ctrl Pts',(-21.2097371145961,18.8725531087288,
-1.27395610155824));
#117654=CARTESIAN_POINT('Ctrl Pts',(-20.358641983851,21.1095172903669,-1.40113190823968));
#117655=CARTESIAN_POINT('Ctrl Pts',(-18.0170393638344,21.6046935058561,
-1.52830771492111));
#117656=CARTESIAN_POINT('Ctrl Pts',(-16.333203267628,19.9038128993918,-1.65548352160254));
#117657=CARTESIAN_POINT('Ctrl Pts',(-16.8519493500829,17.5673150993311,
-1.78265932828398));
#117658=CARTESIAN_POINT('Ctrl Pts',(-19.0973599935785,16.7387984392048,
-1.90983513496541));
#117659=CARTESIAN_POINT('Ctrl Pts',(-21.0094104459781,18.1783720950554,
-2.03701094164685));
#117660=CARTESIAN_POINT('Ctrl Pts',(-20.8339130159653,20.5653183707664,
-2.16418674832828));
#117661=CARTESIAN_POINT('Ctrl Pts',(-18.7318757426636,21.7097612836464,
-2.29136255500972));
#117662=CARTESIAN_POINT('Ctrl Pts',(-16.6317873365857,20.561745973449,-2.41853836169115));
#117663=CARTESIAN_POINT('Ctrl Pts',(-16.4603485748086,18.1745049842297,
-2.54571416837258));
#117664=CARTESIAN_POINT('Ctrl Pts',(-18.3748438750272,16.7381838840222,
-2.67288997505402));
#117665=CARTESIAN_POINT('Ctrl Pts',(-20.6188426291484,17.5705180670209,
-2.80006578173545));
#117666=CARTESIAN_POINT('Ctrl Pts',(-21.1336152570428,19.9078926156331,
-2.92724158841689));
#117667=CARTESIAN_POINT('Ctrl Pts',(-19.4468898237851,21.6059114372621,
-3.05441739509832));
#117668=CARTESIAN_POINT('Ctrl Pts',(-17.1061322239997,21.1067476633747,
-3.18159320177976));
#117669=CARTESIAN_POINT('Ctrl Pts',(-16.2588422718968,18.8683530700484,
-3.30876900846119));
#117670=CARTESIAN_POINT('Ctrl Pts',(-17.6823559096772,16.9443157687486,
-3.43594481514263));
#117671=CARTESIAN_POINT('Ctrl Pts',(-20.0706877279544,17.0998205628843,
-3.56312062182406));
#117672=CARTESIAN_POINT('Ctrl Pts',(-21.2326915200203,19.1922014562322,
-3.6902964285055));
#117673=CARTESIAN_POINT('Ctrl Pts',(-20.102300928759,21.3018288465973,-3.81747223518693));
#117674=CARTESIAN_POINT('Ctrl Pts',(-17.7165791616921,21.4932505417456,
-3.94464804186836));
#117675=CARTESIAN_POINT('Ctrl Pts',(-16.264277865515,19.590849017254,-4.0718238485498));
#117676=CARTESIAN_POINT('Ctrl Pts',(-17.0777933394838,17.3399595955375,
-4.19899965523123));
#117677=CARTESIAN_POINT('Ctrl Pts',(-19.4107756286979,16.8056336150422,
-4.32617546191267));
#117678=CARTESIAN_POINT('Ctrl Pts',(-21.1228582840144,18.4780819988752,
-4.4533512685941));
#117679=CARTESIAN_POINT('Ctrl Pts',(-20.6433117330145,20.8229371587163,
-4.58052707527553));
#117680=CARTESIAN_POINT('Ctrl Pts',(-18.4120901722247,21.6889400235399,
-4.70770288195697));
#117681=CARTESIAN_POINT('Ctrl Pts',(-16.4762008984415,20.281586715068,-4.8348786886384));
#117682=CARTESIAN_POINT('Ctrl Pts',(-16.6117021655217,17.8920365436271,
-4.96205449531983));
#117683=CARTESIAN_POINT('Ctrl Pts',(-18.6942799710763,16.7125534793035,
-5.08923030200127));
#117684=CARTESIAN_POINT('Ctrl Pts',(-20.8132984378653,17.8252400266391,
-5.21640610868271));
#117685=CARTESIAN_POINT('Ctrl Pts',(-21.0246896437286,20.2092753395693,
-5.34358191536413));
#117686=CARTESIAN_POINT('Ctrl Pts',(-19.1345152777048,21.6774549884001,
-5.47075772204558));
#117687=CARTESIAN_POINT('Ctrl Pts',(-16.8768930031683,20.8828152708351,
-5.59793352872701));
#117688=CARTESIAN_POINT('Ctrl Pts',(-16.3230511331653,18.5543888068372,
-5.72510933540844));
#117689=CARTESIAN_POINT('Ctrl Pts',(-17.98110520812,16.8283623586792,-5.85228514208988));
#117690=CARTESIAN_POINT('Ctrl Pts',(-20.3298935247037,17.288258063263,-5.97946094877131));
#117691=CARTESIAN_POINT('Ctrl Pts',(-21.2145485846948,19.5121501559794,
-6.10663675545275));
#117692=CARTESIAN_POINT('Ctrl Pts',(-19.8234542784371,21.4597556720715,
-6.23381256213418));
#117693=CARTESIAN_POINT('Ctrl Pts',(-17.4328532908717,21.3442674325558,
-6.36098836881561));
#117694=CARTESIAN_POINT('Ctrl Pts',(-16.235973650659,19.2716387291798,-6.48816417549706));
#117695=CARTESIAN_POINT('Ctrl Pts',(-17.3308781409654,17.1433777554452,
-6.61533998217847));
#117696=CARTESIAN_POINT('Ctrl Pts',(-19.7130598493718,16.9120318599802,
-6.74251578885992));
#117697=CARTESIAN_POINT('Ctrl Pts',(-21.1970149132871,18.7898465429281,
-6.86969159554135));
#117698=CARTESIAN_POINT('Ctrl Pts',(-20.4213066662076,21.054043383008,-6.99686740222279));
#117699=CARTESIAN_POINT('Ctrl Pts',(-18.0975992789452,21.6273623113514,
-7.12404320890422));
#117700=CARTESIAN_POINT('Ctrl Pts',(-16.3577500537671,19.9838187953891,
-7.25121901558565));
#117701=CARTESIAN_POINT('Ctrl Pts',(-16.7979626675525,17.6312620012014,
-7.37839482226709));
#117702=CARTESIAN_POINT('Ctrl Pts',(-19.0143693698296,16.7280167713133,
-7.50557062894852));
#117703=CARTESIAN_POINT('Ctrl Pts',(-20.9735545769736,18.1027545424254,
-7.63274643562996));
#117704=CARTESIAN_POINT('Ctrl Pts',(-20.8780874621779,20.4942387353917,
-7.75992224231139));
#117705=CARTESIAN_POINT('Ctrl Pts',(-18.8155531779101,21.7084310354144,
-7.88709804899282));
#117706=CARTESIAN_POINT('Ctrl Pts',(-16.6781989146708,20.6313853684961,
-8.01427385567426));
#117707=CARTESIAN_POINT('Ctrl Pts',(-16.4269145498154,18.2512242850411,
-8.1414496623557));
#117708=CARTESIAN_POINT('Ctrl Pts',(-18.2922378916319,16.7515978496617,
-8.26862546903713));
#117709=CARTESIAN_POINT('Ctrl Pts',(-20.5628505490274,17.5083202395048,
-8.39580127571856));
#117710=CARTESIAN_POINT('Ctrl Pts',(-21.155606338957,19.8271456293778,-8.5229770824));
#117711=CARTESIAN_POINT('Ctrl Pts',(-19.5266886147337,21.5806956466073,
-8.65015288908143));
#117712=CARTESIAN_POINT('Ctrl Pts',(-17.1705282862964,21.160196987974,-8.77732869576286));
#117713=CARTESIAN_POINT('Ctrl Pts',(-16.2487562151834,18.9514310736836,
-8.9045045024443));
#117714=CARTESIAN_POINT('Ctrl Pts',(-17.6070410650139,16.9808035386242,
-9.03168030912573));
#117715=CARTESIAN_POINT('Ctrl Pts',(-19.9992407907343,17.0562428352734,
-9.15885611580717));
#117716=CARTESIAN_POINT('Ctrl Pts',(-21.2306606206557,19.1085380912468,
-9.2860319224886));
#117717=CARTESIAN_POINT('Ctrl Pts',(-20.1715492913599,21.2548357889979,
-9.41320772917003));
#117718=CARTESIAN_POINT('Ctrl Pts',(-17.7935757116131,21.5260410050991,
-9.54038353585147));
#117719=CARTESIAN_POINT('Ctrl Pts',(-16.278383047147,19.6733397866716,-9.66755934253291));
#117720=CARTESIAN_POINT('Ctrl Pts',(-17.0160665241465,17.3964705100163,
-9.79473514921434));
#117721=CARTESIAN_POINT('Ctrl Pts',(-19.3298473382647,16.7843194180195,
-9.92191095589577));
#117722=CARTESIAN_POINT('Ctrl Pts',(-21.0969752019817,18.3984971432064,
-10.0490867625772));
#117723=CARTESIAN_POINT('Ctrl Pts',(-20.696219980662,20.7580958098868,-10.1762625692586));
#117724=CARTESIAN_POINT('Ctrl Pts',(-18.4952497161921,21.6983300945914,
-10.3034383759401));
#117725=CARTESIAN_POINT('Ctrl Pts',(-16.5133180186021,20.356593398625,-10.4306141826215));
#117726=CARTESIAN_POINT('Ctrl Pts',(-16.5687242078764,17.9638458629654,
-10.5577899893029));
#117727=CARTESIAN_POINT('Ctrl Pts',(-18.6106365442519,16.7152848409195,
-10.6849657959844));
#117728=CARTESIAN_POINT('Ctrl Pts',(-20.7657271944765,17.7563875757774,
-10.8121416026658));
#117729=CARTESIAN_POINT('Ctrl Pts',(-21.0568342469805,20.1320069264304,
-10.9393174093472));
#117730=CARTESIAN_POINT('Ctrl Pts',(-19.2168850492326,21.6626595862203,
-11.0664932160287));
#117731=CARTESIAN_POINT('Ctrl Pts',(-16.93391879004,20.9440667428082,-11.1936690227101));
#117732=CARTESIAN_POINT('Ctrl Pts',(-16.3024153153455,18.6354927291228,
-11.3208448293915));
#117733=CARTESIAN_POINT('Ctrl Pts',(-17.9017398676552,16.8549109164576,
-11.448020636073));
#117734=CARTESIAN_POINT('Ctrl Pts',(-20.2646114355015,17.2358946025617,
-11.5751964427544));
#117735=CARTESIAN_POINT('Ctrl Pts',(-21.2232420117351,19.428914901949,-11.7023722494359));
#117736=CARTESIAN_POINT('Ctrl Pts',(-19.8981475419851,21.4220118041223,
-11.8295480561173));
#117737=CARTESIAN_POINT('Ctrl Pts',(-17.5050199576091,21.3866426068827,
-11.9567238627987));
#117738=CARTESIAN_POINT('Ctrl Pts',(-16.2394052830226,19.3552563534375,
-12.0838996694802));
#117739=CARTESIAN_POINT('Ctrl Pts',(-17.2624264292529,17.1915238492725,
-12.2110754761616));
#117740=CARTESIAN_POINT('Ctrl Pts',(-19.635524990487,16.880535370574,-12.338251282843));
#117741=CARTESIAN_POINT('Ctrl Pts',(-21.1815303279007,18.707603544426,-12.4654270895244));
#117742=CARTESIAN_POINT('Ctrl Pts',(-20.48207850033,20.9965067219594,-12.5926028962059));
#117743=CARTESIAN_POINT('Ctrl Pts',(-18.1788731466945,21.6473183031405,
-12.7197787028873));
#117744=CARTESIAN_POINT('Ctrl Pts',(-16.3849622259084,20.0629590561579,
-12.8469545095688));
#117745=CARTESIAN_POINT('Ctrl Pts',(-16.7461476651242,17.6969802536931,
-12.9741303162502));
#117746=CARTESIAN_POINT('Ctrl Pts',(-18.9310642415578,16.7200205978014,
-13.1013061229316));
#117747=CARTESIAN_POINT('Ctrl Pts',(-20.9351866075484,18.0283799358088,
-13.2284819296131));
#117748=CARTESIAN_POINT('Ctrl Pts',(-20.9198568821621,20.4217197810322,
-13.3556577362945));
#117749=CARTESIAN_POINT('Ctrl Pts',(-18.8991391369708,21.7042993729031,
-13.4828335429759));
#117750=CARTESIAN_POINT('Ctrl Pts',(-16.7269164832995,20.6994315417472,
-13.6100093496574));
#117751=CARTESIAN_POINT('Ctrl Pts',(-16.3960683825486,18.3290201535185,
-13.7371851563388));
#117752=CARTESIAN_POINT('Ctrl Pts',(-18.2101274324079,16.7677705325936,
-13.8643609630202));
#117753=CARTESIAN_POINT('Ctrl Pts',(-20.5048070478343,17.4480323040911,
-13.9915367697017));
#117754=CARTESIAN_POINT('Ctrl Pts',(-21.1748811055536,19.7457075144692,
-14.1187125763831));
#117755=CARTESIAN_POINT('Ctrl Pts',(-19.6055982470946,21.5528217680131,
-14.2458883830645));
#117756=CARTESIAN_POINT('Ctrl Pts',(-17.2366780944146,21.2114598992563,
-14.373064189746));
#117757=CARTESIAN_POINT('Ctrl Pts',(-16.2414578558307,19.0348002354761,
-14.5002399964274));
#117758=CARTESIAN_POINT('Ctrl Pts',(-17.5329903299092,17.0197929194559,
-14.6274158031088));
#117759=CARTESIAN_POINT('Ctrl Pts',(-19.926374633229,17.0150820981853,-14.7545916097903));
#117760=CARTESIAN_POINT('Ctrl Pts',(-21.2258292176773,19.0249896577937,
-14.8817674164717));
#117761=CARTESIAN_POINT('Ctrl Pts',(-20.2391851552704,21.2055501612724,
-15.0089432231531));
#117762=CARTESIAN_POINT('Ctrl Pts',(-17.8716271352296,21.5562346875283,
-15.1361190298346));
#117763=CARTESIAN_POINT('Ctrl Pts',(-16.2952426937192,19.7553119496581,
-15.263294836516));
#117764=CARTESIAN_POINT('Ctrl Pts',(-16.956266714372,17.4550167817861,-15.3904706431974));
#117765=CARTESIAN_POINT('Ctrl Pts',(-19.2482506860169,16.7657272280153,
-15.5176464498789));
#117766=CARTESIAN_POINT('Ctrl Pts',(-21.0684415712385,18.3198236717957,
-15.6448222565603));
#117767=CARTESIAN_POINT('Ctrl Pts',(-20.7469272066334,20.6915190840625,
-15.7719980632418));
#117768=CARTESIAN_POINT('Ctrl Pts',(-18.5786770662948,21.7049301280797,
-15.8991738699232));
#117769=CARTESIAN_POINT('Ctrl Pts',(-16.5529260772022,20.4303150703446,
-16.0263496766046));
#117770=CARTESIAN_POINT('Ctrl Pts',(-16.5281750395616,18.0370541147968,
-16.153525483286));
#117771=CARTESIAN_POINT('Ctrl Pts',(-18.5271314941858,16.7208156456237,
-16.2807012899675));
#117772=CARTESIAN_POINT('Ctrl Pts',(-20.7158769631869,17.689166763319,-16.4078770966489));
#117773=CARTESIAN_POINT('Ctrl Pts',(-21.0863733276212,20.0537054200458,
-16.5350529033304));
#117774=CARTESIAN_POINT('Ctrl Pts',(-19.2987131687179,21.6451141580778,
-16.6622287100118));
#117775=CARTESIAN_POINT('Ctrl Pts',(-16.9929637275681,21.0033742342365,
-16.7894045166932));
#117776=CARTESIAN_POINT('Ctrl Pts',(-16.2845070054764,18.7172421977746,
-16.9165803233747));
#117777=CARTESIAN_POINT('Ctrl Pts',(-17.8233080731787,16.884102298789,-17.0437561300561));
#117778=CARTESIAN_POINT('Ctrl Pts',(-20.1976124598239,17.1857466171053,
-17.1709319367376));
#117779=CARTESIAN_POINT('Ctrl Pts',(-21.2291432566148,19.3454352128261,
-17.2981077434189));
#117780=CARTESIAN_POINT('Ctrl Pts',(-19.9715349815179,21.3817878447692,
-17.4252835501004));
#117781=CARTESIAN_POINT('Ctrl Pts',(-17.5785651709616,21.4265773634257,
-17.5524593567818));
#117782=CARTESIAN_POINT('Ctrl Pts',(-16.245635101675,19.4387121653785,-17.6796351634633));
#117783=CARTESIAN_POINT('Ctrl Pts',(-17.195625381257,17.2419351890085,-17.8068109701447));
#117784=CARTESIAN_POINT('Ctrl Pts',(-19.5569788912398,16.8516529627759,
-17.9339867768261));
#117785=CARTESIAN_POINT('Ctrl Pts',(-21.1633003483382,18.6259252056079,
-18.0611625835076));
#117786=CARTESIAN_POINT('Ctrl Pts',(-20.5408895152254,20.9369672584502,
-18.188338390189));
#117787=CARTESIAN_POINT('Ctrl Pts',(-18.2607697000954,21.6645414772881,
-18.3155141968704));
#117788=CARTESIAN_POINT('Ctrl Pts',(-16.4148093131604,20.1411436746453,
-18.4426900035519));
#117789=CARTESIAN_POINT('Ctrl Pts',(-16.696562436159,17.7643967817956,-18.5698658102333));
#117790=CARTESIAN_POINT('Ctrl Pts',(-18.8475380664095,16.7148185552248,
-18.6970416169147));
#117791=CARTESIAN_POINT('Ctrl Pts',(-20.8943495675715,17.955331873938,-18.8242174235962));
#117792=CARTESIAN_POINT('Ctrl Pts',(-20.9591744271437,20.3478427623818,
-18.9513932302776));
#117793=CARTESIAN_POINT('Ctrl Pts',(-18.9825398592484,21.6973709774882,
-19.078569036959));
#117794=CARTESIAN_POINT('Ctrl Pts',(-16.77788539751,20.7658081409326,-19.2057448436405));
#117795=CARTESIAN_POINT('Ctrl Pts',(-16.3678446716688,18.4078053400529,
-19.3329206503219));
#117796=CARTESIAN_POINT('Ctrl Pts',(-18.1286046027284,16.7866837825795,
-19.4600964570034));
#117797=CARTESIAN_POINT('Ctrl Pts',(-20.4447772293123,17.3897218945994,
-19.5872722636848));
#117798=CARTESIAN_POINT('Ctrl Pts',(-21.1914179431377,19.6636696077008,
-19.7144480703662));
#117799=CARTESIAN_POINT('Ctrl Pts',(-19.683530194942,21.5223210888799,-19.8416238770476));
#117800=CARTESIAN_POINT('Ctrl Pts',(-17.3045074731465,21.2604788559019,
-19.9687996837291));
#117801=CARTESIAN_POINT('Ctrl Pts',(-16.2369553322288,19.118367116143,-20.0959754904105));
#117802=CARTESIAN_POINT('Ctrl Pts',(-17.4602868598787,17.0612400309757,
-20.223151297092));
#117803=CARTESIAN_POINT('Ctrl Pts',(-19.8521708105233,16.9763848025611,
-20.3503271037734));
#117804=CARTESIAN_POINT('Ctrl Pts',(-21.2182030751438,18.9416493308234,
-20.4775029104549));
#117805=CARTESIAN_POINT('Ctrl Pts',(-20.305131989166,21.154028290157,-20.6046787171362));
#117806=CARTESIAN_POINT('Ctrl Pts',(-17.9506471621875,21.5837957108187,
-20.7318545238177));
#117807=CARTESIAN_POINT('Ctrl Pts',(-16.3148354273652,19.8366774312875,
-20.8590303304991));
#117808=CARTESIAN_POINT('Ctrl Pts',(-16.8984657403956,17.5155252757358,
-20.9862061371806));
#117809=CARTESIAN_POINT('Ctrl Pts',(-19.1660680401668,16.7498922826988,
-21.113381943862));
#117810=CARTESIAN_POINT('Ctrl Pts',(-21.0373070469929,18.2421221167019,
-21.2405577505435));
#117811=CARTESIAN_POINT('Ctrl Pts',(-20.7953425225475,20.6233350697589,
-21.3677335572248));
#117812=CARTESIAN_POINT('Ctrl Pts',(-18.6623441810672,21.7086297969706,
-21.4949093639063));
#117813=CARTESIAN_POINT('Ctrl Pts',(-16.5948543422637,20.502867400276,-21.6220851705877));
#117814=CARTESIAN_POINT('Ctrl Pts',(-16.4903436183303,18.1111966683195,
-21.7492609772692));
#117815=CARTESIAN_POINT('Ctrl Pts',(-18.4433885098623,16.7298792897364,
-21.8764367839506));
#117816=CARTESIAN_POINT('Ctrl Pts',(-20.6647168984764,17.6222041838633,
-22.003612590632));
#117817=CARTESIAN_POINT('Ctrl Pts',(-21.1114420608105,19.9774734447106,
-22.1307883973135));
#117818=CARTESIAN_POINT('Ctrl Pts',(-19.9599075668543,21.0705044715179,
-22.2155722684344));
#117819=CARTESIAN_POINT('Ctrl Pts',(-19.2802415985968,21.2523731445725,
-22.2579642039949));
#117820=CARTESIAN_POINT('Ctrl Pts',(-17.0028273852109,20.6688092100886,
0.0844763361257092));
#117821=CARTESIAN_POINT('Ctrl Pts',(-16.5172190142843,20.092181868941,0.0420657430668536));
#117822=CARTESIAN_POINT('Ctrl Pts',(-16.1763706746349,18.4257326299315,
-0.0427367855524801));
#117823=CARTESIAN_POINT('Ctrl Pts',(-18.01364439973,16.6318023132686,-0.169931249732292));
#117824=CARTESIAN_POINT('Ctrl Pts',(-20.5111535200096,17.2110802832593,
-0.297107056413726));
#117825=CARTESIAN_POINT('Ctrl Pts',(-21.3783870101994,19.6218281451444,
-0.424282863095161));
#117826=CARTESIAN_POINT('Ctrl Pts',(-19.8194850134989,21.6573811366705,
-0.551458669776596));
#117827=CARTESIAN_POINT('Ctrl Pts',(-17.2647560862599,21.4476431456228,
-0.678634476458029));
#117828=CARTESIAN_POINT('Ctrl Pts',(-16.057947487624,19.1863846079818,-0.805810283139464));
#117829=CARTESIAN_POINT('Ctrl Pts',(-17.3062612289062,16.947470098725,-0.932986089820897));
#117830=CARTESIAN_POINT('Ctrl Pts',(-19.8644313564054,16.7853278416859,
-1.06016189650233));
#117831=CARTESIAN_POINT('Ctrl Pts',(-21.3855036379843,18.848524857474,-1.18733770318377));
#117832=CARTESIAN_POINT('Ctrl Pts',(-20.4739844697589,21.2443037270014,
-1.3145135098652));
#117833=CARTESIAN_POINT('Ctrl Pts',(-17.9661382896929,21.774635291315,-1.44168931654664));
#117834=CARTESIAN_POINT('Ctrl Pts',(-16.1627571841069,19.9529995896776,
-1.56886512322807));
#117835=CARTESIAN_POINT('Ctrl Pts',(-16.7183319730092,17.4506206494911,
-1.69604092990951));
#117836=CARTESIAN_POINT('Ctrl Pts',(-19.1231569662995,16.5632829246964,
-1.82321673659094));
#117837=CARTESIAN_POINT('Ctrl Pts',(-21.1709546507375,18.1050600233756,
-1.95039254327237));
#117838=CARTESIAN_POINT('Ctrl Pts',(-20.9829976696055,20.6614690606707,
-2.07756834995381));
#117839=CARTESIAN_POINT('Ctrl Pts',(-18.7317249296694,21.8871624224887,
-2.20474415663524));
#117840=CARTESIAN_POINT('Ctrl Pts',(-16.4825394180193,20.6576430387449,
-2.33191996331668));
#117841=CARTESIAN_POINT('Ctrl Pts',(-16.2989292528432,18.1009183645693,
-2.45909576999811));
#117842=CARTESIAN_POINT('Ctrl Pts',(-18.3493453586185,16.5626247387795,
-2.58627157667954));
#117843=CARTESIAN_POINT('Ctrl Pts',(-20.7526582245547,17.4540510138992,
-2.71344738336098));
#117844=CARTESIAN_POINT('Ctrl Pts',(-21.3039774609752,19.9573689479556,
-2.84062319004241));
#117845=CARTESIAN_POINT('Ctrl Pts',(-19.4975018880252,21.7759396905319,
-2.96779899672385));
#117846=CARTESIAN_POINT('Ctrl Pts',(-16.9905607209365,21.2413374685879,
-3.09497480340528));
#117847=CARTESIAN_POINT('Ctrl Pts',(-16.0831168824194,18.8440266343892,
-3.22215061008672));
#117848=CARTESIAN_POINT('Ctrl Pts',(-17.6076937718807,16.7833910871266,
-3.34932641676815));
#117849=CARTESIAN_POINT('Ctrl Pts',(-20.1655867192137,16.9499360425438,
-3.47650222344959));
#117850=CARTESIAN_POINT('Ctrl Pts',(-21.4100877059499,19.1908668417195,
-3.60367803013102));
#117851=CARTESIAN_POINT('Ctrl Pts',(-20.1994443192179,21.4502685638837,
-3.73085383681246));
#117852=CARTESIAN_POINT('Ctrl Pts',(-17.6443467253329,21.6552803634332,
-3.85802964349388));
#117853=CARTESIAN_POINT('Ctrl Pts',(-16.0889383794468,19.6178166386469,
-3.98520545017533));
#117854=CARTESIAN_POINT('Ctrl Pts',(-16.9602098993781,17.2071238978084,
-4.11238125685675));
#117855=CARTESIAN_POINT('Ctrl Pts',(-19.4588237428005,16.6348631061435,
-4.23955706353819));
#117856=CARTESIAN_POINT('Ctrl Pts',(-21.2924567898383,18.4260480215086,
-4.36673287021963));
#117857=CARTESIAN_POINT('Ctrl Pts',(-20.7788645279368,20.9373776575228,
-4.49390867690106));
#117858=CARTESIAN_POINT('Ctrl Pts',(-18.3892359802594,21.8648629438428,
-4.62108448358249));
#117859=CARTESIAN_POINT('Ctrl Pts',(-16.3159070222257,20.3575936964975,
-4.74826029026393));
#117860=CARTESIAN_POINT('Ctrl Pts',(-16.4610282875234,17.7983958982468,
-4.87543609694536));
#117861=CARTESIAN_POINT('Ctrl Pts',(-18.6914600224833,16.535174687256,-5.0026119036268));
#117862=CARTESIAN_POINT('Ctrl Pts',(-20.9609195464861,17.7268571202586,
-5.12978771030823));
#117863=CARTESIAN_POINT('Ctrl Pts',(-21.1873186048029,20.280148529128,-5.25696351698966));
#117864=CARTESIAN_POINT('Ctrl Pts',(-19.1629501133386,21.8525625213641,
-5.38413932367111));
#117865=CARTESIAN_POINT('Ctrl Pts',(-16.7450465165327,21.0015068541093,
-5.51131513035253));
#117866=CARTESIAN_POINT('Ctrl Pts',(-16.1518842924324,18.5077722795978,
-5.63849093703398));
#117867=CARTESIAN_POINT('Ctrl Pts',(-17.9276529658501,16.6592054913206,
-5.7656667437154));
#117868=CARTESIAN_POINT('Ctrl Pts',(-20.4431949955591,17.1517517825272,
-5.89284255039684));
#117869=CARTESIAN_POINT('Ctrl Pts',(-21.390656701448,19.5335305019064,-6.02001835707826));
#117870=CARTESIAN_POINT('Ctrl Pts',(-19.9008007744696,21.6194075042871,
-6.14719416375971));
#117871=CARTESIAN_POINT('Ctrl Pts',(-17.3404775567387,21.4957201041125,
-6.27436997044113));
#117872=CARTESIAN_POINT('Ctrl Pts',(-16.0586246889428,19.2759438141371,
-6.40154577712258));
#117873=CARTESIAN_POINT('Ctrl Pts',(-17.2312626165228,16.9965856055586,
-6.528721583804));
#117874=CARTESIAN_POINT('Ctrl Pts',(-19.7825688230421,16.7488151618222,
-6.65589739048545));
#117875=CARTESIAN_POINT('Ctrl Pts',(-21.3718782159412,18.7599464866879,
-6.78307319716687));
#117876=CARTESIAN_POINT('Ctrl Pts',(-20.5410980709011,21.1848914144791,
-6.91024900384832));
#117877=CARTESIAN_POINT('Ctrl Pts',(-18.0524176069647,21.7989134830039,
-7.03742481052974));
#117878=CARTESIAN_POINT('Ctrl Pts',(-16.189046684864,20.0386855548983,-7.16460061721119));
#117879=CARTESIAN_POINT('Ctrl Pts',(-16.6605124717835,17.5191075021328,
-7.2917764238926));
#117880=CARTESIAN_POINT('Ctrl Pts',(-19.0342743706914,16.551735805469,-7.41895223057406));
#117881=CARTESIAN_POINT('Ctrl Pts',(-21.1325531716193,18.024073954737,-7.54612803725548));
#117882=CARTESIAN_POINT('Ctrl Pts',(-21.0303083085858,20.5853430815951,
-7.67330384393691));
#117883=CARTESIAN_POINT('Ctrl Pts',(-18.8213430973923,21.8857377324416,
-7.80047965061835));
#117884=CARTESIAN_POINT('Ctrl Pts',(-16.5322460154652,20.7322265267193,
-7.92765545729978));
#117885=CARTESIAN_POINT('Ctrl Pts',(-16.2631215580847,18.1830844006987,
-8.05483126398122));
#117886=CARTESIAN_POINT('Ctrl Pts',(-18.2608747111494,16.5769910373997,
-8.18200707066265));
#117887=CARTESIAN_POINT('Ctrl Pts',(-20.6926909512673,17.3874374122526,
-8.30918287734408));
#117888=CARTESIAN_POINT('Ctrl Pts',(-21.3275298136684,19.8708892783049,
-8.43635868402552));
#117889=CARTESIAN_POINT('Ctrl Pts',(-19.5829660446433,21.7489336888602,
-8.56353449070696));
#117890=CARTESIAN_POINT('Ctrl Pts',(-17.0595286224332,21.2985814618163,
-8.69071029738838));
#117891=CARTESIAN_POINT('Ctrl Pts',(-16.0723147597259,18.9330028134741,
-8.81788610406983));
#117892=CARTESIAN_POINT('Ctrl Pts',(-17.5270319021526,16.8224693293182,
-8.94506191075126));
#117893=CARTESIAN_POINT('Ctrl Pts',(-20.0890673614655,16.90326448658,-9.07223771743269));
#117894=CARTESIAN_POINT('Ctrl Pts',(-21.4079126215994,19.1012637431849,
-9.19941352411413));
#117895=CARTESIAN_POINT('Ctrl Pts',(-20.2736090131502,21.3999392044174,
-9.32658933079555));
#117896=CARTESIAN_POINT('Ctrl Pts',(-17.726809694048,21.6903988064862,-9.453765137477));
#117897=CARTESIAN_POINT('Ctrl Pts',(-16.1040449673761,19.7061638924493,
-9.58094094415843));
#117898=CARTESIAN_POINT('Ctrl Pts',(-16.894100749718,17.2676468404274,-9.70811675083986));
#117899=CARTESIAN_POINT('Ctrl Pts',(-19.3721498971671,16.6120356942131,
-9.83529255752129));
#117900=CARTESIAN_POINT('Ctrl Pts',(-21.2647361220149,18.3408129886411,
-9.96246836420274));
#117901=CARTESIAN_POINT('Ctrl Pts',(-20.8355290301125,20.8679328560937,
-10.0896441708842));
#117902=CARTESIAN_POINT('Ctrl Pts',(-18.4782994886839,21.8749196689318,
-10.2168199775656));
#117903=CARTESIAN_POINT('Ctrl Pts',(-16.3556592958241,20.4379255270265,
-10.3439957842471));
#117904=CARTESIAN_POINT('Ctrl Pts',(-16.4149990825736,17.875303365661,-10.4711715909285));
#117905=CARTESIAN_POINT('Ctrl Pts',(-18.6018782776321,16.5380999636187,
-10.59834739761));
#117906=CARTESIAN_POINT('Ctrl Pts',(-20.9099709525642,17.65311644607,-10.7255232042914));
#117907=CARTESIAN_POINT('Ctrl Pts',(-21.2217453345073,20.1973943960938,
-10.8526990109728));
#117908=CARTESIAN_POINT('Ctrl Pts',(-19.2511677789294,21.8367167102424,
-10.9798748176543));
#117909=CARTESIAN_POINT('Ctrl Pts',(-16.806120885236,21.0671069131022,-11.1070506243357));
#117910=CARTESIAN_POINT('Ctrl Pts',(-16.1297834216659,18.5946342261783,
-11.2342264310171));
#117911=CARTESIAN_POINT('Ctrl Pts',(-17.8426530328072,16.6876388807614,
-11.3614022376985));
#117912=CARTESIAN_POINT('Ctrl Pts',(-20.3732781631159,17.0956707447917,
-11.48857804438));
#117913=CARTESIAN_POINT('Ctrl Pts',(-21.3999673238431,19.4443859083351,
-11.6157538510614));
#117914=CARTESIAN_POINT('Ctrl Pts',(-19.9807969335377,21.5789839865442,
-11.7429296577429));
#117915=CARTESIAN_POINT('Ctrl Pts',(-17.4177677416566,21.5411037307608,
-11.8701054644243));
#117916=CARTESIAN_POINT('Ctrl Pts',(-16.062299952218,19.3654979245523,-11.9972812711057));
#117917=CARTESIAN_POINT('Ctrl Pts',(-17.157951132213,17.0481498617898,-12.1244570777871));
#117918=CARTESIAN_POINT('Ctrl Pts',(-19.6995293277776,16.7150825592159,
-12.2516328844686));
#117919=CARTESIAN_POINT('Ctrl Pts',(-21.3552942926149,18.671864594454,-12.37880869115));
#117920=CARTESIAN_POINT('Ctrl Pts',(-20.6061844398505,21.1232699017635,
-12.5059844978315));
#117921=CARTESIAN_POINT('Ctrl Pts',(-18.1394615643946,21.8202862630607,
-12.6331603045129));
#117922=CARTESIAN_POINT('Ctrl Pts',(-16.2181908023896,20.1234444285697,
-12.7603361111943));
#117923=CARTESIAN_POINT('Ctrl Pts',(-16.605018830463,17.5894914635544,-12.8875119178758));
#117924=CARTESIAN_POINT('Ctrl Pts',(-18.9450549421127,16.5431719385577,
-13.0146877245572));
#117925=CARTESIAN_POINT('Ctrl Pts',(-21.091461243921,17.9444190758505,-13.1418635312386));
#117926=CARTESIAN_POINT('Ctrl Pts',(-21.0750431749784,20.5076755981723,
-13.2690393379201));
#117927=CARTESIAN_POINT('Ctrl Pts',(-18.9108632945195,21.8813127399352,
-13.3962151446015));
#117928=CARTESIAN_POINT('Ctrl Pts',(-16.5844223187131,20.8051036811079,
-13.5233909512829));
#117929=CARTESIAN_POINT('Ctrl Pts',(-16.2300854476496,18.2664034360971,
-13.6505667579644));
#117930=CARTESIAN_POINT('Ctrl Pts',(-18.1729347679036,16.5943119101923,
-13.7777425646458));
#117931=CARTESIAN_POINT('Ctrl Pts',(-20.6305266149702,17.3228692967068,
-13.9049183713272));
#117932=CARTESIAN_POINT('Ctrl Pts',(-21.3481730045189,19.7836694128848,
-14.0320941780087));
#117933=CARTESIAN_POINT('Ctrl Pts',(-19.6674779162968,21.7190808866133,
-14.1592699846901));
#117934=CARTESIAN_POINT('Ctrl Pts',(-17.1303747780463,21.3534838159302,
-14.2864457913715));
#117935=CARTESIAN_POINT('Ctrl Pts',(-16.0644982487317,19.0222908216738,
-14.413621598053));
#117936=CARTESIAN_POINT('Ctrl Pts',(-17.447723888241,16.8642267859192,-14.5407974047344));
#117937=CARTESIAN_POINT('Ctrl Pts',(-20.0110280249899,16.859181516911,-14.6679732114158));
#117938=CARTESIAN_POINT('Ctrl Pts',(-21.4027382101088,19.0117837358195,
-14.7951490180973));
#117939=CARTESIAN_POINT('Ctrl Pts',(-20.3460467280269,21.3471545123578,
-14.9223248247787));
#117940=CARTESIAN_POINT('Ctrl Pts',(-17.8104024278843,21.7227361085096,
-15.0495006314601));
#117941=CARTESIAN_POINT('Ctrl Pts',(-16.1221015752275,19.7939557210286,
-15.1766764381416));
#117942=CARTESIAN_POINT('Ctrl Pts',(-16.8300554146003,17.3303496418165,
-15.303852244823));
#117943=CARTESIAN_POINT('Ctrl Pts',(-19.284760238949,16.5921235399122,-15.4310280515045));
#117944=CARTESIAN_POINT('Ctrl Pts',(-21.2341767280976,18.2565540443337,
-15.5582038581859));
#117945=CARTESIAN_POINT('Ctrl Pts',(-20.8898362476853,20.7966294734819,
-15.6853796648673));
#117946=CARTESIAN_POINT('Ctrl Pts',(-18.5676498163098,21.8819882759749,
-15.8125554715487));
#117947=CARTESIAN_POINT('Ctrl Pts',(-16.3980793536131,20.5168811154897,
-15.9397312782302));
#117948=CARTESIAN_POINT('Ctrl Pts',(-16.3715711003901,17.9537090836658,
-16.0669070849116));
#117949=CARTESIAN_POINT('Ctrl Pts',(-18.5124447336848,16.5440234313033,
-16.1940828915931));
#117950=CARTESIAN_POINT('Ctrl Pts',(-20.8565815725531,17.5811232494858,
-16.3212586982745));
#117951=CARTESIAN_POINT('Ctrl Pts',(-21.253381560874,20.1135338247049,-16.4484345049559));
#117952=CARTESIAN_POINT('Ctrl Pts',(-19.338805337548,21.8179256333241,-16.5756103116374));
#117953=CARTESIAN_POINT('Ctrl Pts',(-16.8693577554744,21.1306249774212,
-16.7027861183188));
#117954=CARTESIAN_POINT('Ctrl Pts',(-16.1106037000031,18.6821875500976,
-16.8299619250002));
#117955=CARTESIAN_POINT('Ctrl Pts',(-17.7586529234411,16.7189027237572,
-16.9571377316817));
#117956=CARTESIAN_POINT('Ctrl Pts',(-20.3015225527551,17.0419624713682,
-17.0843135383631));
#117957=CARTESIAN_POINT('Ctrl Pts',(-21.4062875313382,19.354979525847,-17.2114893450445));
#117958=CARTESIAN_POINT('Ctrl Pts',(-20.0593945607884,21.5359043017382,
-17.338665151726));
#117959=CARTESIAN_POINT('Ctrl Pts',(-17.4965343439791,21.5838736806199,
-17.4658409584074));
#117960=CARTESIAN_POINT('Ctrl Pts',(-16.0689720607886,19.4548787346826,
-17.5930167650888));
#117961=CARTESIAN_POINT('Ctrl Pts',(-17.0864075015351,17.1021401864965,
-17.7201925717703));
#117962=CARTESIAN_POINT('Ctrl Pts',(-19.6154067985012,16.684149626596,-17.8473683784517));
#117963=CARTESIAN_POINT('Ctrl Pts',(-21.3357700641153,18.584387450276,-17.9745441851331));
#117964=CARTESIAN_POINT('Ctrl Pts',(-20.6691707799709,21.0595033963588,
-18.1017199918146));
#117965=CARTESIAN_POINT('Ctrl Pts',(-18.2271724154379,21.8387322073577,
-18.228895798496));
#117966=CARTESIAN_POINT('Ctrl Pts',(-16.2501569024917,20.207179813531,-18.3560716051774));
#117967=CARTESIAN_POINT('Ctrl Pts',(-16.5519132667841,17.6616942707386,
-18.4832474118589));
#117968=CARTESIAN_POINT('Ctrl Pts',(-18.8555987732945,16.537600573676,-18.6104232185403));
#117969=CARTESIAN_POINT('Ctrl Pts',(-21.0477249524445,17.8661849205939,
-18.7375990252217));
#117970=CARTESIAN_POINT('Ctrl Pts',(-21.1171520939507,20.4285536338248,
-18.8647748319032));
#117971=CARTESIAN_POINT('Ctrl Pts',(-19.0001851038609,21.8738924587027,
-18.9919506385846));
#117972=CARTESIAN_POINT('Ctrl Pts',(-16.639009803247,20.8761927289634,-19.119126445266));
#117973=CARTESIAN_POINT('Ctrl Pts',(-16.1998579765528,18.3507820268139,
-19.2463022519475));
#117974=CARTESIAN_POINT('Ctrl Pts',(-18.0856241733337,16.6145679183314,
-19.3734780586289));
#117975=CARTESIAN_POINT('Ctrl Pts',(-20.5662349414884,17.2604191027876,
-19.5006538653103));
#117976=CARTESIAN_POINT('Ctrl Pts',(-21.3658838853536,19.695807173002,-19.6278296719918));
#117977=CARTESIAN_POINT('Ctrl Pts',(-19.7509426921062,21.6864147924606,
-19.7550054786732));
#117978=CARTESIAN_POINT('Ctrl Pts',(-17.2030197464517,21.4059829044279,
-19.8821812853547));
#117979=CARTESIAN_POINT('Ctrl Pts',(-16.059676065617,19.1117905859247,-20.0093570920361));
#117980=CARTESIAN_POINT('Ctrl Pts',(-17.3698587893405,16.908616461354,-20.1365328987175));
#117981=CARTESIAN_POINT('Ctrl Pts',(-19.9315560549264,16.8177368822917,
-20.2637087053989));
#117982=CARTESIAN_POINT('Ctrl Pts',(-21.3945706447594,18.9225266095884,
-20.3908845120804));
#117983=CARTESIAN_POINT('Ctrl Pts',(-20.4166754991338,21.2919748133934,
-20.5180603187618));
#117984=CARTESIAN_POINT('Ctrl Pts',(-17.8950325316693,21.7522538440923,
-20.6452361254433));
#117985=CARTESIAN_POINT('Ctrl Pts',(-16.1430853073993,19.881097796524,-20.7724119321247));
#117986=CARTESIAN_POINT('Ctrl Pts',(-16.7681508238931,17.395153974591,-20.8995877388061));
#117987=CARTESIAN_POINT('Ctrl Pts',(-19.1967429841419,16.5751643826307,
-21.0267635454876));
#117988=CARTESIAN_POINT('Ctrl Pts',(-21.2008317885977,18.1733360181572,
-21.153939352169));
#117989=CARTESIAN_POINT('Ctrl Pts',(-20.9416888395956,20.7236046919281,
-21.2811151588505));
#117990=CARTESIAN_POINT('Ctrl Pts',(-18.6572569308498,21.8859506052002,
-21.4082909655318));
#117991=CARTESIAN_POINT('Ctrl Pts',(-16.4429843423899,20.5945843440041,
-21.5354667722133));
#117992=CARTESIAN_POINT('Ctrl Pts',(-16.3310538134642,18.033115434702,-21.6626425788947));
#117993=CARTESIAN_POINT('Ctrl Pts',(-18.4227563631869,16.5537305545665,
-21.7898183855762));
#117994=CARTESIAN_POINT('Ctrl Pts',(-20.8017893666684,17.50940661932,-21.9169941922576));
#117995=CARTESIAN_POINT('Ctrl Pts',(-21.2802300646426,20.0318897120323,
-22.0441699989391));
#117996=CARTESIAN_POINT('Ctrl Pts',(-20.0469416504615,21.2025211683863,
-22.12895387006));
#117997=CARTESIAN_POINT('Ctrl Pts',(-19.3190223666151,21.3973017229923,
-22.1713458056205));
#117998=CARTESIAN_POINT('Ctrl Pts',(-16.8880690316762,20.7654464739225,
0.171094734500185));
#117999=CARTESIAN_POINT('Ctrl Pts',(-16.3702699845374,20.1505948657621,
0.128684141441329));
#118000=CARTESIAN_POINT('Ctrl Pts',(-16.006827020915,18.3736777454539,0.043881612821995));
#118001=CARTESIAN_POINT('Ctrl Pts',(-17.9658924760107,16.4608289063181,
-0.0833128513578171));
#118002=CARTESIAN_POINT('Ctrl Pts',(-20.6289599190898,17.0785068518555,
-0.210488658039252));
#118003=CARTESIAN_POINT('Ctrl Pts',(-21.5536817767679,19.6490616868026,
-0.337664464720685));
#118004=CARTESIAN_POINT('Ctrl Pts',(-19.8914411384235,21.8195502173065,
-0.46484027140212));
#118005=CARTESIAN_POINT('Ctrl Pts',(-17.1673608230486,21.5959088255693,
-0.592016078083554));
#118006=CARTESIAN_POINT('Ctrl Pts',(-15.8805536346544,19.1847528689885,
-0.719191884764988));
#118007=CARTESIAN_POINT('Ctrl Pts',(-17.2116173157294,16.7974221125058,
-0.846367691446423));
#118008=CARTESIAN_POINT('Ctrl Pts',(-19.9393669463845,16.6245315463164,
-0.973543498127856));
#118009=CARTESIAN_POINT('Ctrl Pts',(-21.5612701613726,18.8244966062191,
-1.10071930480929));
#118010=CARTESIAN_POINT('Ctrl Pts',(-20.5893269556668,21.379090163636,-1.22789511149073));
#118011=CARTESIAN_POINT('Ctrl Pts',(-17.9152372155514,21.9445770767739,
-1.35507091817216));
#118012=CARTESIAN_POINT('Ctrl Pts',(-15.9923111005858,20.0021862799634,
-1.4822467248536));
#118013=CARTESIAN_POINT('Ctrl Pts',(-16.5847145959355,17.3339261996511,
-1.60942253153503));
#118014=CARTESIAN_POINT('Ctrl Pts',(-19.1489539390206,16.3877674101879,
-1.73659833821646));
#118015=CARTESIAN_POINT('Ctrl Pts',(-21.332498855497,18.0317479516957,-1.8637741448979));
#118016=CARTESIAN_POINT('Ctrl Pts',(-21.1320823232458,20.7576197505752,
-1.99094995157933));
#118017=CARTESIAN_POINT('Ctrl Pts',(-18.7315741166753,22.064563561331,-2.11812575826077));
#118018=CARTESIAN_POINT('Ctrl Pts',(-16.3332914994529,20.7535401040407,
-2.2453015649422));
#118019=CARTESIAN_POINT('Ctrl Pts',(-16.1375099308779,18.0273317449088,
-2.37247737162363));
#118020=CARTESIAN_POINT('Ctrl Pts',(-18.3238468422098,16.387065593537,-2.49965317830507));
#118021=CARTESIAN_POINT('Ctrl Pts',(-20.8864738199611,17.3375839607775,
-2.62682898498651));
#118022=CARTESIAN_POINT('Ctrl Pts',(-21.4743396649076,20.006845280278,-2.75400479166794));
#118023=CARTESIAN_POINT('Ctrl Pts',(-19.5481139522653,21.9459679438018,
-2.88118059834937));
#118024=CARTESIAN_POINT('Ctrl Pts',(-16.8749892178732,21.3759272738012,
-3.00835640503081));
#118025=CARTESIAN_POINT('Ctrl Pts',(-15.9073914929419,18.8197001987301,
-3.13553221171224));
#118026=CARTESIAN_POINT('Ctrl Pts',(-17.5330316340844,16.6224664055047,
-3.26270801839368));
#118027=CARTESIAN_POINT('Ctrl Pts',(-20.2604857104729,16.8000515222033,
-3.38988382507511));
#118028=CARTESIAN_POINT('Ctrl Pts',(-21.5874838918795,19.1895322272068,
-3.51705963175655));
#118029=CARTESIAN_POINT('Ctrl Pts',(-20.2965877096769,21.5987082811702,
-3.64423543843798));
#118030=CARTESIAN_POINT('Ctrl Pts',(-17.5721142889738,21.8173101851209,
-3.77141124511941));
#118031=CARTESIAN_POINT('Ctrl Pts',(-15.9135988933785,19.64478426004,-3.89858705180085));
#118032=CARTESIAN_POINT('Ctrl Pts',(-16.8426264592725,17.0742882000792,
-4.02576285848228));
#118033=CARTESIAN_POINT('Ctrl Pts',(-19.5068718569032,16.4640925972449,
-4.15293866516372));
#118034=CARTESIAN_POINT('Ctrl Pts',(-21.4620552956622,18.3740140441421,
-4.28011447184515));
#118035=CARTESIAN_POINT('Ctrl Pts',(-20.914417322859,21.0518181563291,-4.40729027852659));
#118036=CARTESIAN_POINT('Ctrl Pts',(-18.3663817882941,22.0407858641459,
-4.53446608520802));
#118037=CARTESIAN_POINT('Ctrl Pts',(-16.15561314601,20.4336006779268,-4.66164189188945));
#118038=CARTESIAN_POINT('Ctrl Pts',(-16.3103544095251,17.7047552528665,
-4.78881769857089));
#118039=CARTESIAN_POINT('Ctrl Pts',(-18.6886400738904,16.3577958952085,
-4.91599350525232));
#118040=CARTESIAN_POINT('Ctrl Pts',(-21.1085406551067,17.628474213878,-5.04316931193375));
#118041=CARTESIAN_POINT('Ctrl Pts',(-21.3499475658771,20.3510217186868,
-5.1703451186152));
#118042=CARTESIAN_POINT('Ctrl Pts',(-19.1913849489723,22.0276700543283,
-5.29752092529662));
#118043=CARTESIAN_POINT('Ctrl Pts',(-16.613200029897,21.1201984373834,-5.42469673197806));
#118044=CARTESIAN_POINT('Ctrl Pts',(-15.9807174516997,18.4611557523585,
-5.5518725386595));
#118045=CARTESIAN_POINT('Ctrl Pts',(-17.8742007235803,16.4900486239617,
-5.67904834534092));
#118046=CARTESIAN_POINT('Ctrl Pts',(-20.5564964664144,17.0152455017915,
-5.80622415202237));
#118047=CARTESIAN_POINT('Ctrl Pts',(-21.5667648182011,19.5549108478334,
-5.93339995870379));
#118048=CARTESIAN_POINT('Ctrl Pts',(-19.9781472705019,21.7790593365027,
-6.06057576538524));
#118049=CARTESIAN_POINT('Ctrl Pts',(-17.2481018226055,21.6471727756692,
-6.18775157206665));
#118050=CARTESIAN_POINT('Ctrl Pts',(-15.8812757272267,19.2802488990946,
-6.31492737874811));
#118051=CARTESIAN_POINT('Ctrl Pts',(-17.1316470920802,16.849793455672,-6.44210318542952));
#118052=CARTESIAN_POINT('Ctrl Pts',(-19.8520777967125,16.5855984636642,
-6.56927899211098));
#118053=CARTESIAN_POINT('Ctrl Pts',(-21.5467415185955,18.7300464304477,
-6.6964547987924));
#118054=CARTESIAN_POINT('Ctrl Pts',(-20.6608894755945,21.3157394459503,
-6.82363060547384));
#118055=CARTESIAN_POINT('Ctrl Pts',(-18.0072359349844,21.9704646546564,
-6.95080641215527));
#118056=CARTESIAN_POINT('Ctrl Pts',(-16.020343315961,20.0935523144076,-7.07798221883671));
#118057=CARTESIAN_POINT('Ctrl Pts',(-16.5230622760143,17.4069530030642,
-7.20515802551813));
#118058=CARTESIAN_POINT('Ctrl Pts',(-19.0541793715532,16.3754548396247,
-7.33233383219958));
#118059=CARTESIAN_POINT('Ctrl Pts',(-21.291551766265,17.9453933670485,-7.459509638881));
#118060=CARTESIAN_POINT('Ctrl Pts',(-21.1825291549937,20.6764474277986,
-7.58668544556244));
#118061=CARTESIAN_POINT('Ctrl Pts',(-18.8271330168744,22.0630444294688,
-7.71386125224388));
#118062=CARTESIAN_POINT('Ctrl Pts',(-16.3862931162597,20.8330676849425,
-7.84103705892531));
#118063=CARTESIAN_POINT('Ctrl Pts',(-16.099328566354,18.1149445163563,-7.96821286560675));
#118064=CARTESIAN_POINT('Ctrl Pts',(-18.2295115306668,16.4023842251376,
-8.09538867228817));
#118065=CARTESIAN_POINT('Ctrl Pts',(-20.8225313535071,17.2665545850003,
-8.22256447896962));
#118066=CARTESIAN_POINT('Ctrl Pts',(-21.4994532883798,19.9146329272319,
-8.34974028565105));
#118067=CARTESIAN_POINT('Ctrl Pts',(-19.6392434745528,21.917171731113,-8.47691609233248));
#118068=CARTESIAN_POINT('Ctrl Pts',(-16.9485289585702,21.4369659356584,
-8.60409189901392));
#118069=CARTESIAN_POINT('Ctrl Pts',(-15.8958733042685,18.9145745532647,
-8.73126770569535));
#118070=CARTESIAN_POINT('Ctrl Pts',(-17.4470227392911,16.6641351200123,
-8.85844351237678));
#118071=CARTESIAN_POINT('Ctrl Pts',(-20.1788939321968,16.7502861378866,
-8.98561931905823));
#118072=CARTESIAN_POINT('Ctrl Pts',(-21.5851646225432,19.093989395123,-9.11279512573965));
#118073=CARTESIAN_POINT('Ctrl Pts',(-20.3756687349405,21.5450426198368,
-9.23997093242109));
#118074=CARTESIAN_POINT('Ctrl Pts',(-17.6600436764829,21.8547566078734,
-9.36714673910252));
#118075=CARTESIAN_POINT('Ctrl Pts',(-15.9297068876053,19.738987998227,-9.49432254578396));
#118076=CARTESIAN_POINT('Ctrl Pts',(-16.7721349752896,17.1388231708385,
-9.62149835246539));
#118077=CARTESIAN_POINT('Ctrl Pts',(-19.4144524560694,16.4397519704066,
-9.74867415914682));
#118078=CARTESIAN_POINT('Ctrl Pts',(-21.432497042048,18.2831288340757,-9.87584996582827));
#118079=CARTESIAN_POINT('Ctrl Pts',(-20.974838079563,20.9777699023008,-10.0030257725097));
#118080=CARTESIAN_POINT('Ctrl Pts',(-18.4613492611758,22.0515092432722,
-10.1302015791911));
#118081=CARTESIAN_POINT('Ctrl Pts',(-16.1980005730462,20.5192576554282,
-10.2573773858725));
#118082=CARTESIAN_POINT('Ctrl Pts',(-16.2612739572708,17.7867608683564,
-10.384553192554));
#118083=CARTESIAN_POINT('Ctrl Pts',(-18.5931200110123,16.3609150863178,
-10.5117289992354));
#118084=CARTESIAN_POINT('Ctrl Pts',(-21.0542147106519,17.5498453163626,
-10.6389048059168));
#118085=CARTESIAN_POINT('Ctrl Pts',(-21.3866564220343,20.2627818657572,
-10.7660806125983));
#118086=CARTESIAN_POINT('Ctrl Pts',(-19.2854505086261,22.0107738342645,
-10.8932564192797));
#118087=CARTESIAN_POINT('Ctrl Pts',(-16.6783229804319,21.1901470833962,
-11.0204322259611));
#118088=CARTESIAN_POINT('Ctrl Pts',(-15.9571515279862,18.5537757232337,
-11.1476080326426));
#118089=CARTESIAN_POINT('Ctrl Pts',(-17.7835661979594,16.5203668450652,
-11.274783839324));
#118090=CARTESIAN_POINT('Ctrl Pts',(-20.4819448907301,16.9554468870216,
-11.4019596460055));
#118091=CARTESIAN_POINT('Ctrl Pts',(-21.5766926359512,19.4598569147211,
-11.5291354526869));
#118092=CARTESIAN_POINT('Ctrl Pts',(-20.0634463250904,21.735956168966,-11.6563112593683));
#118093=CARTESIAN_POINT('Ctrl Pts',(-17.330515525704,21.6955648546388,-11.7834870660497));
#118094=CARTESIAN_POINT('Ctrl Pts',(-15.8851946214135,19.3757394956669,
-11.9106628727312));
#118095=CARTESIAN_POINT('Ctrl Pts',(-17.053475835173,16.9047758743069,-12.0378386794126));
#118096=CARTESIAN_POINT('Ctrl Pts',(-19.7635336650682,16.5496297478578,
-12.165014486094));
#118097=CARTESIAN_POINT('Ctrl Pts',(-21.5290582573291,18.6361256444822,
-12.2921902927755));
#118098=CARTESIAN_POINT('Ctrl Pts',(-20.7302903793709,21.2500330815675,
-12.4193660994569));
#118099=CARTESIAN_POINT('Ctrl Pts',(-18.1000499820946,21.9932542229807,
-12.5465419061383));
#118100=CARTESIAN_POINT('Ctrl Pts',(-16.0514193788707,20.1839298009815,
-12.6737177128198));
#118101=CARTESIAN_POINT('Ctrl Pts',(-16.4638899958019,17.4820026734157,
-12.8008935195012));
#118102=CARTESIAN_POINT('Ctrl Pts',(-18.9590456426675,16.3663232793141,
-12.9280693261827));
#118103=CARTESIAN_POINT('Ctrl Pts',(-21.2477358802935,17.8604582158923,
-13.0552451328641));
#118104=CARTESIAN_POINT('Ctrl Pts',(-21.2302294677946,20.5936314153126,
-13.1824209395455));
#118105=CARTESIAN_POINT('Ctrl Pts',(-18.9225874520683,22.0583261069674,
-13.309596746227));
#118106=CARTESIAN_POINT('Ctrl Pts',(-16.4419281541264,20.9107758204687,
-13.4367725529084));
#118107=CARTESIAN_POINT('Ctrl Pts',(-16.0641025127507,18.2037867186756,
-13.5639483595899));
#118108=CARTESIAN_POINT('Ctrl Pts',(-18.1357421033992,16.4208532877909,
-13.6911241662712));
#118109=CARTESIAN_POINT('Ctrl Pts',(-20.756246182106,17.1977062893226,-13.8182999729527));
#118110=CARTESIAN_POINT('Ctrl Pts',(-21.5214649034841,19.8216313113002,
-13.9454757796341));
#118111=CARTESIAN_POINT('Ctrl Pts',(-19.7293575854992,21.8853400052135,
-14.0726515863156));
#118112=CARTESIAN_POINT('Ctrl Pts',(-17.0240714616778,21.495507732604,-14.199827392997));
#118113=CARTESIAN_POINT('Ctrl Pts',(-15.8875386416327,19.0097814078715,
-14.3270031996784));
#118114=CARTESIAN_POINT('Ctrl Pts',(-17.3624574465728,16.7086606523826,
-14.4541790063599));
#118115=CARTESIAN_POINT('Ctrl Pts',(-20.0956814167509,16.7032809356367,
-14.5813548130413));
#118116=CARTESIAN_POINT('Ctrl Pts',(-21.5796472025402,18.9985778138453,
-14.7085306197227));
#118117=CARTESIAN_POINT('Ctrl Pts',(-20.4529083007835,21.4887588634431,
-14.8357064264042));
#118118=CARTESIAN_POINT('Ctrl Pts',(-17.749177720539,21.8892375294908,-14.9628822330856));
#118119=CARTESIAN_POINT('Ctrl Pts',(-15.9489604567358,19.8325994923992,
-15.090058039767));
#118120=CARTESIAN_POINT('Ctrl Pts',(-16.7038441148285,17.2056825018467,
-15.2172338464485));
#118121=CARTESIAN_POINT('Ctrl Pts',(-19.321269791881,16.4185198518092,-15.3444096531299));
#118122=CARTESIAN_POINT('Ctrl Pts',(-21.3999118849568,18.1932844168717,
-15.4715854598113));
#118123=CARTESIAN_POINT('Ctrl Pts',(-21.0327452887372,20.9017398629015,
-15.5987612664928));
#118124=CARTESIAN_POINT('Ctrl Pts',(-18.5566225663247,22.05904642387,-15.7259370731742));
#118125=CARTESIAN_POINT('Ctrl Pts',(-16.2432326300242,20.6034471606347,
-15.8531128798556));
#118126=CARTESIAN_POINT('Ctrl Pts',(-16.2149671612184,17.8703640525348,
-15.9802886865371));
#118127=CARTESIAN_POINT('Ctrl Pts',(-18.4977579731839,16.367231216983,-16.1074644932185));
#118128=CARTESIAN_POINT('Ctrl Pts',(-20.9972861819192,17.4730797356526,
-16.2346402999));
#118129=CARTESIAN_POINT('Ctrl Pts',(-21.4203897941269,20.1733622293642,
-16.3618161065814));
#118130=CARTESIAN_POINT('Ctrl Pts',(-19.378897506378,21.9907371085704,-16.4889919132628));
#118131=CARTESIAN_POINT('Ctrl Pts',(-16.7457517833806,21.2578757206061,
-16.6161677199442));
#118132=CARTESIAN_POINT('Ctrl Pts',(-15.9367003945299,18.6471329024206,
-16.7433435266257));
#118133=CARTESIAN_POINT('Ctrl Pts',(-17.6939977737036,16.5537031487253,
-16.8705193333071));
#118134=CARTESIAN_POINT('Ctrl Pts',(-20.4054326456863,16.8981783256312,
-16.9976951399886));
#118135=CARTESIAN_POINT('Ctrl Pts',(-21.5834318060615,19.364523838868,-17.12487094667));
#118136=CARTESIAN_POINT('Ctrl Pts',(-20.1472541400588,21.6900207587073,
-17.2520467533514));
#118137=CARTESIAN_POINT('Ctrl Pts',(-17.4145035169965,21.7411699978141,
-17.3792225600329));
#118138=CARTESIAN_POINT('Ctrl Pts',(-15.8923090199021,19.4710453039867,
-17.5063983667143));
#118139=CARTESIAN_POINT('Ctrl Pts',(-16.9771896218132,16.9623451839844,
-17.6335741733957));
#118140=CARTESIAN_POINT('Ctrl Pts',(-19.6738347057625,16.5166462904161,
-17.7607499800772));
#118141=CARTESIAN_POINT('Ctrl Pts',(-21.5082397798925,18.542849694944,-17.8879257867586));
#118142=CARTESIAN_POINT('Ctrl Pts',(-20.7974520447164,21.1820395342675,
-18.01510159344));
#118143=CARTESIAN_POINT('Ctrl Pts',(-18.1935751307804,22.0129229374273,
-18.1422774001214));
#118144=CARTESIAN_POINT('Ctrl Pts',(-16.085504491823,20.2732159524167,-18.2694532068029));
#118145=CARTESIAN_POINT('Ctrl Pts',(-16.4072640974092,17.5589917596816,
-18.3966290134843));
#118146=CARTESIAN_POINT('Ctrl Pts',(-18.8636594801795,16.3603825921271,
-18.5238048201658));
#118147=CARTESIAN_POINT('Ctrl Pts',(-21.2011003373174,17.7770379672497,
-18.6509806268472));
#118148=CARTESIAN_POINT('Ctrl Pts',(-21.2751297607577,20.5092645052679,
-18.7781564335287));
#118149=CARTESIAN_POINT('Ctrl Pts',(-19.0178303484736,22.0504139399173,
-18.90533224021));
#118150=CARTESIAN_POINT('Ctrl Pts',(-16.5001342089838,20.9865773169943,
-19.0325080468915));
#118151=CARTESIAN_POINT('Ctrl Pts',(-16.0318712814367,18.2937587135751,
-19.1596838535729));
#118152=CARTESIAN_POINT('Ctrl Pts',(-18.042643743939,16.4424520540833,-19.2868596602544));
#118153=CARTESIAN_POINT('Ctrl Pts',(-20.6876926536642,17.1311163109758,
-19.4140354669358));
#118154=CARTESIAN_POINT('Ctrl Pts',(-21.5403498275698,19.7279447383034,
-19.5412112736172));
#118155=CARTESIAN_POINT('Ctrl Pts',(-19.8183551892704,21.8505084960413,
-19.6683870802987));
#118156=CARTESIAN_POINT('Ctrl Pts',(-17.1015320197568,21.5514869529538,
-19.7955628869801));
#118157=CARTESIAN_POINT('Ctrl Pts',(-15.8823967990051,19.1052140557062,
-19.9227386936616));
#118158=CARTESIAN_POINT('Ctrl Pts',(-17.2794307188022,16.7559928917323,
-20.049914500343));
#118159=CARTESIAN_POINT('Ctrl Pts',(-20.0109412993294,16.6590889620223,
-20.1770903070244));
#118160=CARTESIAN_POINT('Ctrl Pts',(-21.5709382143749,18.9034038883535,
-20.3042661137059));
#118161=CARTESIAN_POINT('Ctrl Pts',(-20.5282190091016,21.4299213366298,
-20.4314419203873));
#118162=CARTESIAN_POINT('Ctrl Pts',(-17.839417901151,21.920711977366,-20.5586177270687));
#118163=CARTESIAN_POINT('Ctrl Pts',(-15.9713351874334,19.9255181617605,
-20.6857935337502));
#118164=CARTESIAN_POINT('Ctrl Pts',(-16.6378359073908,17.2747826734461,
-20.8129693404316));
#118165=CARTESIAN_POINT('Ctrl Pts',(-19.227417928117,16.4004364825627,-20.940145147113));
#118166=CARTESIAN_POINT('Ctrl Pts',(-21.3643565302024,18.1045499196127,
-21.0673209537945));
#118167=CARTESIAN_POINT('Ctrl Pts',(-21.0880351566437,20.8238743140973,
-21.1944967604759));
#118168=CARTESIAN_POINT('Ctrl Pts',(-18.6521696806325,22.0632714134299,
-21.3216725671574));
#118169=CARTESIAN_POINT('Ctrl Pts',(-16.2911143425161,20.6863012877323,
-21.4488483738387));
#118170=CARTESIAN_POINT('Ctrl Pts',(-16.171764008598,17.9550342010845,-21.5760241805202));
#118171=CARTESIAN_POINT('Ctrl Pts',(-18.4021242165115,16.3775818193965,
-21.7031999872016));
#118172=CARTESIAN_POINT('Ctrl Pts',(-20.9388618348603,17.3966090547766,
-21.8303757938831));
#118173=CARTESIAN_POINT('Ctrl Pts',(-21.4490180684747,20.086305979354,-21.9575516005645));
#118174=CARTESIAN_POINT('Ctrl Pts',(-20.1339757340687,21.3345378652548,
-22.0423354716855));
#118175=CARTESIAN_POINT('Ctrl Pts',(-19.3578031346334,21.5422303014122,
-22.0847274072459));
#118176=CARTESIAN_POINT('Ctrl Pts',(-16.7733106781415,20.8620837377565,
0.257713132874659));
#118177=CARTESIAN_POINT('Ctrl Pts',(-16.2233209547904,20.2090078625832,
0.215302539815803));
#118178=CARTESIAN_POINT('Ctrl Pts',(-15.8372833671953,18.3216228609763,
0.13050001119647));
#118179=CARTESIAN_POINT('Ctrl Pts',(-17.9181405522913,16.2898554993676,
0.00330554701665787));
#118180=CARTESIAN_POINT('Ctrl Pts',(-20.7467663181702,16.9459334204518,
-0.123870259664777));
#118181=CARTESIAN_POINT('Ctrl Pts',(-21.7289765433362,19.6762952284609,
-0.251046066346211));
#118182=CARTESIAN_POINT('Ctrl Pts',(-19.9633972633481,21.9817192979427,
-0.378221873027645));
#118183=CARTESIAN_POINT('Ctrl Pts',(-17.0699655598372,21.7441745055157,
-0.50539767970908));
#118184=CARTESIAN_POINT('Ctrl Pts',(-15.703159781685,19.1831211299953,-0.632573486390514));
#118185=CARTESIAN_POINT('Ctrl Pts',(-17.1169734025524,16.6473741262867,
-0.759749293071947));
#118186=CARTESIAN_POINT('Ctrl Pts',(-20.0143025363638,16.4637352509469,
-0.886925099753383));
#118187=CARTESIAN_POINT('Ctrl Pts',(-21.7370366847608,18.8004683549644,
-1.01410090643482));
#118188=CARTESIAN_POINT('Ctrl Pts',(-20.7046694415748,21.5138766002705,
-1.14127671311625));
#118189=CARTESIAN_POINT('Ctrl Pts',(-17.8643361414099,22.1145188622328,
-1.26845251979769));
#118190=CARTESIAN_POINT('Ctrl Pts',(-15.8218650170646,20.0513729702491,
-1.39562832647912));
#118191=CARTESIAN_POINT('Ctrl Pts',(-16.4510972188617,17.217231749811,-1.52280413316055));
#118192=CARTESIAN_POINT('Ctrl Pts',(-19.1747509117416,16.2122518956796,
-1.64997993984199));
#118193=CARTESIAN_POINT('Ctrl Pts',(-21.4940430602564,17.9584358800158,
-1.77715574652343));
#118194=CARTESIAN_POINT('Ctrl Pts',(-21.281166976886,20.8537704404796,-1.90433155320486));
#118195=CARTESIAN_POINT('Ctrl Pts',(-18.7314233036813,22.2419647001733,
-2.03150735988629));
#118196=CARTESIAN_POINT('Ctrl Pts',(-16.1840435808866,20.8494371693366,
-2.15868316656773));
#118197=CARTESIAN_POINT('Ctrl Pts',(-15.9760906089126,17.9537451252482,
-2.28585897324916));
#118198=CARTESIAN_POINT('Ctrl Pts',(-18.2983483258012,16.2115064482945,
-2.4130347799306));
#118199=CARTESIAN_POINT('Ctrl Pts',(-21.0202894153674,17.2211169076559,
-2.54021058661203));
#118200=CARTESIAN_POINT('Ctrl Pts',(-21.64470186884,20.0563216126004,-2.66738639329346));
#118201=CARTESIAN_POINT('Ctrl Pts',(-19.5987260165054,22.1159961970718,
-2.7945621999749));
#118202=CARTESIAN_POINT('Ctrl Pts',(-16.75941771481,21.5105170790144,-2.92173800665633));
#118203=CARTESIAN_POINT('Ctrl Pts',(-15.7316661034645,18.7953737630709,
-3.04891381333777));
#118204=CARTESIAN_POINT('Ctrl Pts',(-17.4583694962879,16.4615417238828,
-3.1760896200192));
#118205=CARTESIAN_POINT('Ctrl Pts',(-20.3553847017321,16.6501670018626,
-3.30326542670064));
#118206=CARTESIAN_POINT('Ctrl Pts',(-21.7648800778091,19.1881976126941,
-3.43044123338207));
#118207=CARTESIAN_POINT('Ctrl Pts',(-20.3937311001358,21.7471479984566,
-3.5576170400635));
#118208=CARTESIAN_POINT('Ctrl Pts',(-17.4998818526146,21.9793400068086,
-3.68479284674494));
#118209=CARTESIAN_POINT('Ctrl Pts',(-15.7382594073102,19.671751881433,-3.81196865342637));
#118210=CARTESIAN_POINT('Ctrl Pts',(-16.7250430191669,16.9414525023501,
-3.93914446010781));
#118211=CARTESIAN_POINT('Ctrl Pts',(-19.5549199710057,16.2933220883461,
-4.06632026678924));
#118212=CARTESIAN_POINT('Ctrl Pts',(-21.6316538014862,18.3219800667756,
-4.19349607347067));
#118213=CARTESIAN_POINT('Ctrl Pts',(-21.0499701177813,21.1662586551355,
-4.32067188015211));
#118214=CARTESIAN_POINT('Ctrl Pts',(-18.3435275963289,22.2167087844487,
-4.44784768683354));
#118215=CARTESIAN_POINT('Ctrl Pts',(-15.995319269794,20.5096076593562,-4.57502349351498));
#118216=CARTESIAN_POINT('Ctrl Pts',(-16.1596805315267,17.6111146074862,
-4.70219930019641));
#118217=CARTESIAN_POINT('Ctrl Pts',(-18.6858201252975,16.180417103161,-4.82937510687785));
#118218=CARTESIAN_POINT('Ctrl Pts',(-21.2561617637276,17.5300913074975,
-4.95655091355928));
#118219=CARTESIAN_POINT('Ctrl Pts',(-21.5125765269513,20.4218949082454,
-5.08372672024072));
#118220=CARTESIAN_POINT('Ctrl Pts',(-19.2198197846062,22.2027775872924,
-5.21090252692215));
#118221=CARTESIAN_POINT('Ctrl Pts',(-16.4813535432613,21.2388900206576,
-5.33807833360358));
#118222=CARTESIAN_POINT('Ctrl Pts',(-15.8095506109669,18.4145392251191,
-5.46525414028503));
#118223=CARTESIAN_POINT('Ctrl Pts',(-17.8207484813105,16.3208917566031,
-5.59242994696645));
#118224=CARTESIAN_POINT('Ctrl Pts',(-20.6697979372697,16.8787392210558,
-5.71960575364789));
#118225=CARTESIAN_POINT('Ctrl Pts',(-21.7428729349543,19.5762911937604,
-5.84678156032932));
#118226=CARTESIAN_POINT('Ctrl Pts',(-20.0554937665343,21.9387111687183,
-5.97395736701076));
#118227=CARTESIAN_POINT('Ctrl Pts',(-17.1557260884723,21.7986254472259,
-6.10113317369219));
#118228=CARTESIAN_POINT('Ctrl Pts',(-15.7039267655104,19.284553984052,-6.22830898037363));
#118229=CARTESIAN_POINT('Ctrl Pts',(-17.0320315676376,16.7030013057854,
-6.35548478705506));
#118230=CARTESIAN_POINT('Ctrl Pts',(-19.9215867703828,16.4223817655062,
-6.48266059373649));
#118231=CARTESIAN_POINT('Ctrl Pts',(-21.7216048212496,18.7001463742074,
-6.60983640041793));
#118232=CARTESIAN_POINT('Ctrl Pts',(-20.7806808802879,21.4465874774214,
-6.73701220709936));
#118233=CARTESIAN_POINT('Ctrl Pts',(-17.9620542630039,22.1420158263089,
-6.8641880137808));
#118234=CARTESIAN_POINT('Ctrl Pts',(-15.8516399470578,20.1484190739168,
-6.99136382046223));
#118235=CARTESIAN_POINT('Ctrl Pts',(-16.3856120802451,17.2947985039956,
-7.11853962714367));
#118236=CARTESIAN_POINT('Ctrl Pts',(-19.0740843724149,16.1991738737805,
-7.2457154338251));
#118237=CARTESIAN_POINT('Ctrl Pts',(-21.4505503609105,17.86671277936,-7.37289124050654));
#118238=CARTESIAN_POINT('Ctrl Pts',(-21.3347500014016,20.7675517740021,
-7.50006704718796));
#118239=CARTESIAN_POINT('Ctrl Pts',(-18.8329229363566,22.240351126496,-7.62724285386941));
#118240=CARTESIAN_POINT('Ctrl Pts',(-16.2403402170543,20.9339088431657,
-7.75441866055083));
#118241=CARTESIAN_POINT('Ctrl Pts',(-15.9355355746231,18.0468046320139,
-7.88159446723227));
#118242=CARTESIAN_POINT('Ctrl Pts',(-18.1981483501842,16.2277774128756,
-8.0087702739137));
#118243=CARTESIAN_POINT('Ctrl Pts',(-20.952371755747,17.145671757748,-8.13594608059513));
#118244=CARTESIAN_POINT('Ctrl Pts',(-21.6713767630913,19.958376576159,-8.26312188727658));
#118245=CARTESIAN_POINT('Ctrl Pts',(-19.6955209044624,22.0854097733659,
-8.390297693958));
#118246=CARTESIAN_POINT('Ctrl Pts',(-16.8375292947071,21.5753504095007,
-8.51747350063944));
#118247=CARTESIAN_POINT('Ctrl Pts',(-15.719431848811,18.8961462930551,-8.64464930732087));
#118248=CARTESIAN_POINT('Ctrl Pts',(-17.3670135764298,16.5058009107065,
-8.77182511400231));
#118249=CARTESIAN_POINT('Ctrl Pts',(-20.268720502928,16.5973077891932,-8.89900092068374));
#118250=CARTESIAN_POINT('Ctrl Pts',(-21.7624166234869,19.0867150470611,
-9.02617672736517));
#118251=CARTESIAN_POINT('Ctrl Pts',(-20.4777284567308,21.6901460352563,
-9.15335253404662));
#118252=CARTESIAN_POINT('Ctrl Pts',(-17.5932776589179,22.0191144092604,
-9.28052834072804));
#118253=CARTESIAN_POINT('Ctrl Pts',(-15.7553688078344,19.7718121040047,
-9.40770414740949));
#118254=CARTESIAN_POINT('Ctrl Pts',(-16.6501692008611,17.0099995012495,
-9.53487995409091));
#118255=CARTESIAN_POINT('Ctrl Pts',(-19.4567550149717,16.2674682466002,
-9.66205576077236));
#118256=CARTESIAN_POINT('Ctrl Pts',(-21.6002579620812,18.2254446795103,
-9.78923156745378));
#118257=CARTESIAN_POINT('Ctrl Pts',(-21.1141471290137,21.0876069485077,
-9.91640737413522));
#118258=CARTESIAN_POINT('Ctrl Pts',(-18.4443990336675,22.2280988176125,
-10.0435831808167));
#118259=CARTESIAN_POINT('Ctrl Pts',(-16.0403418502683,20.6005897838297,
-10.1707589874981));
#118260=CARTESIAN_POINT('Ctrl Pts',(-16.1075488319678,17.698218371052,-10.2979347941796));
#118261=CARTESIAN_POINT('Ctrl Pts',(-18.5843617443927,16.183730209017,-10.425110600861));
#118262=CARTESIAN_POINT('Ctrl Pts',(-21.1984584687395,17.4465741866552,
-10.5522864075424));
#118263=CARTESIAN_POINT('Ctrl Pts',(-21.5515675095613,20.3281693354206,
-10.6794622142238));
#118264=CARTESIAN_POINT('Ctrl Pts',(-19.3197332383227,22.1848309582866,
-10.8066380209053));
#118265=CARTESIAN_POINT('Ctrl Pts',(-16.5505250756278,21.3131872536903,
-10.9338138275867));
#118266=CARTESIAN_POINT('Ctrl Pts',(-15.7845196343066,18.5129172202892,
-11.0609896342681));
#118267=CARTESIAN_POINT('Ctrl Pts',(-17.7244793631115,16.3530948093689,
-11.1881654409496));
#118268=CARTESIAN_POINT('Ctrl Pts',(-20.5906116183444,16.8152230292517,
-11.315341247631));
#118269=CARTESIAN_POINT('Ctrl Pts',(-21.7534179480593,19.4753279211071,
-11.4425170543125));
#118270=CARTESIAN_POINT('Ctrl Pts',(-20.1460957166432,21.8929283513879,
-11.5696928609939));
#118271=CARTESIAN_POINT('Ctrl Pts',(-17.2432633097514,21.8500259785168,
-11.6968686676753));
#118272=CARTESIAN_POINT('Ctrl Pts',(-15.7080892906089,19.3859810667816,
-11.8240444743568));
#118273=CARTESIAN_POINT('Ctrl Pts',(-16.9490005381331,16.7614018868241,
-11.9512202810382));
#118274=CARTESIAN_POINT('Ctrl Pts',(-19.8275380023589,16.3841769364998,
-12.0783960877196));
#118275=CARTESIAN_POINT('Ctrl Pts',(-21.7028222220433,18.6003866945102,
-12.205571894401));
#118276=CARTESIAN_POINT('Ctrl Pts',(-20.8543963188915,21.3767962613715,
-12.3327477010825));
#118277=CARTESIAN_POINT('Ctrl Pts',(-18.0606383997947,22.1662221829007,
-12.4599235077639));
#118278=CARTESIAN_POINT('Ctrl Pts',(-15.8846479553519,20.2444151733933,
-12.5870993144454));
#118279=CARTESIAN_POINT('Ctrl Pts',(-16.3227611611408,17.3745138832769,
-12.7142751211268));
#118280=CARTESIAN_POINT('Ctrl Pts',(-18.9730363432223,16.1894746200704,
-12.8414509278082));
#118281=CARTESIAN_POINT('Ctrl Pts',(-21.4040105166661,17.776497355934,-12.9686267344897));
#118282=CARTESIAN_POINT('Ctrl Pts',(-21.385415760611,20.6795872324527,-13.0958025411711));
#118283=CARTESIAN_POINT('Ctrl Pts',(-18.934311609617,22.2353394739996,-13.2229783478525));
#118284=CARTESIAN_POINT('Ctrl Pts',(-16.2994339895399,21.0164479598295,
-13.350154154534));
#118285=CARTESIAN_POINT('Ctrl Pts',(-15.8981195778519,18.1411700012542,
-13.4773299612154));
#118286=CARTESIAN_POINT('Ctrl Pts',(-18.0985494388948,16.2473946653896,
-13.6045057678968));
#118287=CARTESIAN_POINT('Ctrl Pts',(-20.881965749242,17.0725432819383,-13.7316815745783));
#118288=CARTESIAN_POINT('Ctrl Pts',(-21.6947568024494,19.8595932097158,
-13.8588573812597));
#118289=CARTESIAN_POINT('Ctrl Pts',(-19.7912372547015,22.0515991238136,
-13.9860331879411));
#118290=CARTESIAN_POINT('Ctrl Pts',(-16.9177681453095,21.6375316492779,
-14.1132089946226));
#118291=CARTESIAN_POINT('Ctrl Pts',(-15.7105790345338,18.9972719940692,
-14.240384801304));
#118292=CARTESIAN_POINT('Ctrl Pts',(-17.2771910049047,16.5530945188459,
-14.3675606079854));
#118293=CARTESIAN_POINT('Ctrl Pts',(-20.1803348085118,16.5473803543624,
-14.4947364146669));
#118294=CARTESIAN_POINT('Ctrl Pts',(-21.7565561949717,18.9853718918711,
-14.6219122213483));
#118295=CARTESIAN_POINT('Ctrl Pts',(-20.55976987354,21.6303632145285,-14.7490880280298));
#118296=CARTESIAN_POINT('Ctrl Pts',(-17.6879530131938,22.0557389504721,
-14.8762638347112));
#118297=CARTESIAN_POINT('Ctrl Pts',(-15.7758193382441,19.8712432637697,
-15.0034396413926));
#118298=CARTESIAN_POINT('Ctrl Pts',(-16.5776328150568,17.081015361877,-15.130615448074));
#118299=CARTESIAN_POINT('Ctrl Pts',(-19.3577793448131,16.2449161637061,
-15.2577912547555));
#118300=CARTESIAN_POINT('Ctrl Pts',(-21.5656470418159,18.1300147894097,
-15.3849670614369));
#118301=CARTESIAN_POINT('Ctrl Pts',(-21.1756543297891,21.0068502523211,
-15.5121428681183));
#118302=CARTESIAN_POINT('Ctrl Pts',(-18.5455953163398,22.2361045717652,
-15.6393186747998));
#118303=CARTESIAN_POINT('Ctrl Pts',(-16.0883859064352,20.6900132057797,
-15.7664944814812));
#118304=CARTESIAN_POINT('Ctrl Pts',(-16.0583632220467,17.7870190214039,
-15.8936702881626));
#118305=CARTESIAN_POINT('Ctrl Pts',(-18.4830712126828,16.1904390026627,
-16.0208460948441));
#118306=CARTESIAN_POINT('Ctrl Pts',(-21.1379907912855,17.3650362218196,
-16.1480219015255));
#118307=CARTESIAN_POINT('Ctrl Pts',(-21.5873980273797,20.2331906340233,
-16.2751977082069));
#118308=CARTESIAN_POINT('Ctrl Pts',(-19.418989675208,22.1635485838168,-16.4023735148884));
#118309=CARTESIAN_POINT('Ctrl Pts',(-16.622145811287,21.3851264637907,-16.5295493215698));
#118310=CARTESIAN_POINT('Ctrl Pts',(-15.7627970890565,18.6120782547437,
-16.6567251282513));
#118311=CARTESIAN_POINT('Ctrl Pts',(-17.629342623966,16.3885035736934,-16.7839009349327));
#118312=CARTESIAN_POINT('Ctrl Pts',(-20.5093427386175,16.7543941798941,
-16.9110767416142));
#118313=CARTESIAN_POINT('Ctrl Pts',(-21.7605760807848,19.374068151889,-17.0382525482955));
#118314=CARTESIAN_POINT('Ctrl Pts',(-20.2351137193294,21.8441372156765,
-17.165428354977));
#118315=CARTESIAN_POINT('Ctrl Pts',(-17.3324726900139,21.8984663150084,
-17.2926041616584));
#118316=CARTESIAN_POINT('Ctrl Pts',(-15.7156459790158,19.4872118732907,
-17.4197799683399));
#118317=CARTESIAN_POINT('Ctrl Pts',(-16.8679717420912,16.8225501814725,
-17.5469557750213));
#118318=CARTESIAN_POINT('Ctrl Pts',(-19.7322626130239,16.3491429542363,
-17.6741315817028));
#118319=CARTESIAN_POINT('Ctrl Pts',(-21.6807094956696,18.501311939612,-17.8013073883841));
#118320=CARTESIAN_POINT('Ctrl Pts',(-20.925733309462,21.3045756721762,-17.9284831950656));
#118321=CARTESIAN_POINT('Ctrl Pts',(-18.1599778461229,22.1871136674968,
-18.055659001747));
#118322=CARTESIAN_POINT('Ctrl Pts',(-15.9208520811544,20.3392520913025,
-18.1828348084285));
#118323=CARTESIAN_POINT('Ctrl Pts',(-16.2626149280343,17.4562892486245,
-18.3100106151099));
#118324=CARTESIAN_POINT('Ctrl Pts',(-18.8717201870645,16.1831646105782,
-18.4371864217913));
#118325=CARTESIAN_POINT('Ctrl Pts',(-21.3544757221902,17.6878910139056,
-18.5643622284728));
#118326=CARTESIAN_POINT('Ctrl Pts',(-21.4331074275647,20.5899753767109,
-18.6915380351542));
#118327=CARTESIAN_POINT('Ctrl Pts',(-19.0354755930861,22.226935421132,-18.8187138418356));
#118328=CARTESIAN_POINT('Ctrl Pts',(-16.3612586147209,21.0969619050252,
-18.9458896485171));
#118329=CARTESIAN_POINT('Ctrl Pts',(-15.8638845863206,18.2367354003361,
-19.0730654551985));
#118330=CARTESIAN_POINT('Ctrl Pts',(-17.9996633145444,16.2703361898353,
-19.20024126188));
#118331=CARTESIAN_POINT('Ctrl Pts',(-20.8091503658403,17.0018135191641,
-19.3274170685614));
#118332=CARTESIAN_POINT('Ctrl Pts',(-21.7148157697857,19.7600823036045,
-19.4545928752428));
#118333=CARTESIAN_POINT('Ctrl Pts',(-19.8857676864347,22.0146021996221,
-19.5817686819242));
#118334=CARTESIAN_POINT('Ctrl Pts',(-17.000044293062,21.6969910014797,-19.7089444886057));
#118335=CARTESIAN_POINT('Ctrl Pts',(-15.7051175323933,19.0986375254879,
-19.8361202952871));
#118336=CARTESIAN_POINT('Ctrl Pts',(-17.1890026482639,16.6033693221106,
-19.9632961019685));
#118337=CARTESIAN_POINT('Ctrl Pts',(-20.0903265437325,16.500441041753,-20.09047190865));
#118338=CARTESIAN_POINT('Ctrl Pts',(-21.7473057839905,18.8842811671185,
-20.2176477153314));
#118339=CARTESIAN_POINT('Ctrl Pts',(-20.6397625190695,21.5678678598662,
-20.3448235220129));
#118340=CARTESIAN_POINT('Ctrl Pts',(-17.7838032706328,22.0891701106396,
-20.4719993286943));
#118341=CARTESIAN_POINT('Ctrl Pts',(-15.7995850674674,19.9699385269971,
-20.5991751353757));
#118342=CARTESIAN_POINT('Ctrl Pts',(-16.5075209908883,17.1544113723013,
-20.7263509420572));
#118343=CARTESIAN_POINT('Ctrl Pts',(-19.2580928720921,16.2257085824946,
-20.8535267487386));
#118344=CARTESIAN_POINT('Ctrl Pts',(-21.5278812718072,18.035763821068,-20.98070255542));
#118345=CARTESIAN_POINT('Ctrl Pts',(-21.2343814736919,20.9241439362665,
-21.1078783621014));
#118346=CARTESIAN_POINT('Ctrl Pts',(-18.6470824304151,22.2405922216597,
-21.2350541687829));
#118347=CARTESIAN_POINT('Ctrl Pts',(-16.1392443426422,20.7780182314605,
-21.3622299754643));
#118348=CARTESIAN_POINT('Ctrl Pts',(-16.0124742037318,17.8769529674671,
-21.4894057821458));
#118349=CARTESIAN_POINT('Ctrl Pts',(-18.381492069836,16.2014330842265,-21.6165815888272));
#118350=CARTESIAN_POINT('Ctrl Pts',(-21.0759343030523,17.2838114902333,
-21.7437573955087));
#118351=CARTESIAN_POINT('Ctrl Pts',(-21.6178060723068,20.1407222466758,
-21.87093320219));
#118352=CARTESIAN_POINT('Ctrl Pts',(-20.221009817676,21.4665545621232,-21.955717073311));
#118353=CARTESIAN_POINT('Ctrl Pts',(-19.3965839026516,21.687158879832,-21.9981090088715));
#118354=CARTESIAN_POINT('Ctrl Pts',(-17.1140743056112,20.5739122292573,
2.77555756156289E-16));
#118355=CARTESIAN_POINT('Ctrl Pts',(-17.0603911325521,20.522111673172,4.45182444894629E-15));
#118356=CARTESIAN_POINT('Ctrl Pts',(-17.0098645202578,20.4674385257497,
-9.9671288295164E-15));
#118357=CARTESIAN_POINT('Ctrl Pts',(-16.9624881995608,20.410264093257,4.69416172599324E-15));
#118358=CARTESIAN_POINT('Ctrl Pts',(-16.9134245654303,20.3510533863855,
1.9877615930799E-14));
#118359=CARTESIAN_POINT('Ctrl Pts',(-16.8677391100127,20.2891596196004,
4.01703270921356E-15));
#118360=CARTESIAN_POINT('Ctrl Pts',(-16.8254532095188,20.2249455930833,
3.11556336285435E-15));
#118361=CARTESIAN_POINT('Ctrl Pts',(-16.7853187213443,20.1639986330379,
2.25995876655715E-15));
#118362=CARTESIAN_POINT('Ctrl Pts',(-16.7482466106952,20.1009605704099,
1.9879857987986E-14));
#118363=CARTESIAN_POINT('Ctrl Pts',(-16.7142836213594,20.0361088469222,
1.85268467234323E-14));
#118364=CARTESIAN_POINT('Ctrl Pts',(-16.6991853089609,20.0072788881953,
1.79420105219681E-14));
#118365=CARTESIAN_POINT('Ctrl Pts',(-16.6847018341336,19.9780901364722,
-8.23592356720746E-15));
#118366=CARTESIAN_POINT('Ctrl Pts',(-16.6708392964776,19.9485654278612,
1.03597685985335E-14));
#118367=CARTESIAN_POINT('Ctrl Pts',(-16.6640109607001,19.9340223024153,
1.9174859491606E-14));
#118368=CARTESIAN_POINT('Ctrl Pts',(-16.657333302533,19.9193976511972,3.18705451808171E-15));
#118369=CARTESIAN_POINT('Ctrl Pts',(-16.6508071688394,19.9046941363876,
-4.62824223390612E-15));
#118370=CARTESIAN_POINT('Ctrl Pts',(-16.6447949816305,19.8911485536865,
-1.19254541885051E-14));
#118371=CARTESIAN_POINT('Ctrl Pts',(-16.6389109256811,19.8775346474983,
3.85423458197671E-15));
#118372=CARTESIAN_POINT('Ctrl Pts',(-16.6331636045017,19.8638740397009,
6.02989880249538E-15));
#118373=CARTESIAN_POINT('Ctrl Pts',(-16.6020948019513,19.790027683611,1.85394696934408E-14));
#118374=CARTESIAN_POINT('Ctrl Pts',(-16.5749612060018,19.7146929635301,
8.98167354597479E-15));
#118375=CARTESIAN_POINT('Ctrl Pts',(-16.5517844460822,19.6382510185693,
1.35030875370035E-14));
#118376=CARTESIAN_POINT('Ctrl Pts',(-16.5281813102644,19.5604027940833,
1.81076806245845E-14));
#118377=CARTESIAN_POINT('Ctrl Pts',(-16.5086814210928,19.4814054223285,
2.71946254420182E-14));
#118378=CARTESIAN_POINT('Ctrl Pts',(-16.4933485190229,19.4016259047529,
7.14706072102445E-15));
#118379=CARTESIAN_POINT('Ctrl Pts',(-16.4794162838085,19.3291342786354,
-1.10691507889412E-14));
#118380=CARTESIAN_POINT('Ctrl Pts',(-16.4689247639322,19.2559959244269,
1.02006884852949E-14));
#118381=CARTESIAN_POINT('Ctrl Pts',(-16.4619555680579,19.1824703462648,
1.64729341278758E-14));
#118382=CARTESIAN_POINT('Ctrl Pts',(-16.4592976470201,19.1544290650995,
1.9131180430237E-14));
#118383=CARTESIAN_POINT('Ctrl Pts',(-16.4571524088489,19.1263313551069,
2.39160590086535E-14));
#118384=CARTESIAN_POINT('Ctrl Pts',(-16.4555257409501,19.0981913259617,
-4.73232564246473E-15));
#118385=CARTESIAN_POINT('Ctrl Pts',(-16.4546322610198,19.0827348512285,
-2.03445886243926E-14));
#118386=CARTESIAN_POINT('Ctrl Pts',(-16.453895246137,19.0672656072016,-8.75022012521963E-16));
#118387=CARTESIAN_POINT('Ctrl Pts',(-16.4533157740873,19.051785924702,1.26981758441502E-14));
#118388=CARTESIAN_POINT('Ctrl Pts',(-16.4528680721876,19.0398262740765,
2.31564174349633E-14));
#118389=CARTESIAN_POINT('Ctrl Pts',(-16.452514580052,19.0278636904617,5.25880506684687E-15));
#118390=CARTESIAN_POINT('Ctrl Pts',(-16.4522557186358,19.0159077924821,
5.49560397189452E-15));
#118391=CARTESIAN_POINT('Ctrl Pts',(-16.4504488747983,18.9324560332097,
7.08905735160161E-15));
#118392=CARTESIAN_POINT('Ctrl Pts',(-16.4532438607103,18.8492105138102,
6.08038579602206E-16));
#118393=CARTESIAN_POINT('Ctrl Pts',(-16.4606969184041,18.7665518702536,
4.14945855453652E-15));
#118394=CARTESIAN_POINT('Ctrl Pts',(-16.4681357553308,18.6840509430821,
7.10329836543544E-15));
#118395=CARTESIAN_POINT('Ctrl Pts',(-16.4802145308229,18.6021336503298,
7.4706047686461E-15));
#118396=CARTESIAN_POINT('Ctrl Pts',(-16.4970385284052,18.5211628277987,
4.55191440096314E-15));
#118397=CARTESIAN_POINT('Ctrl Pts',(-16.5134762563069,18.4420510505752,
2.05501660863705E-15));
#118398=CARTESIAN_POINT('Ctrl Pts',(-16.5344435942651,18.3638418295306,
-1.67546161971538E-14));
#118399=CARTESIAN_POINT('Ctrl Pts',(-16.5596748813382,18.2867616450374,
-2.91433543964104E-15));
#118400=CARTESIAN_POINT('Ctrl Pts',(-16.5700722924092,18.2549981301094,
2.76440958040333E-15));
#118401=CARTESIAN_POINT('Ctrl Pts',(-16.581194395652,18.2234264109971,1.53541667197338E-14));
#118402=CARTESIAN_POINT('Ctrl Pts',(-16.5930250854222,18.1920628114276,
1.10467190950203E-14));
#118403=CARTESIAN_POINT('Ctrl Pts',(-16.5995763500233,18.1746951647716,
8.82295792525399E-15));
#118404=CARTESIAN_POINT('Ctrl Pts',(-16.6063471420461,18.1573861965041,
1.49165270495576E-14));
#118405=CARTESIAN_POINT('Ctrl Pts',(-16.6133223339605,18.1401687566555,
1.25455201782643E-14));
#118406=CARTESIAN_POINT('Ctrl Pts',(-16.6442815008621,18.0637496988806,
1.85388435652528E-15));
#118407=CARTESIAN_POINT('Ctrl Pts',(-16.6792965711232,17.9890373934243,
2.44510841382609E-16));
#118408=CARTESIAN_POINT('Ctrl Pts',(-16.7180395276146,17.9162554524269,
3.63598040564739E-15));
#118409=CARTESIAN_POINT('Ctrl Pts',(-16.7588464280445,17.8395962170884,
7.20812288916674E-15));
#118410=CARTESIAN_POINT('Ctrl Pts',(-16.8037890252177,17.7650776476886,
-8.42604220156098E-15));
#118411=CARTESIAN_POINT('Ctrl Pts',(-16.8525445311818,17.692966664072,-1.04360964314765E-14));
#118412=CARTESIAN_POINT('Ctrl Pts',(-16.9013000371459,17.6208556804554,
-1.2446150661392E-14));
#118413=CARTESIAN_POINT('Ctrl Pts',(-16.9538690505405,17.5511513968607,
1.86312228584609E-14));
#118414=CARTESIAN_POINT('Ctrl Pts',(-17.0099820350415,17.4841394296583,
-2.55351295663786E-15));
#118415=CARTESIAN_POINT('Ctrl Pts',(-17.0318957421493,17.4579693616242,
-1.0746443255118E-14));
#118416=CARTESIAN_POINT('Ctrl Pts',(-17.0543504737559,17.4322101781547,
-7.53714155281239E-18));
#118417=CARTESIAN_POINT('Ctrl Pts',(-17.0773320757735,17.4068801208169,
7.21644966006352E-16));
#118418=CARTESIAN_POINT('Ctrl Pts',(-17.0864638250902,17.3968152117818,
1.04464455640109E-15));
#118419=CARTESIAN_POINT('Ctrl Pts',(-17.0956795264284,17.3868172601505,
1.08622188611639E-14));
#118420=CARTESIAN_POINT('Ctrl Pts',(-17.1049759845535,17.376889953632,9.32587340685131E-15));
#118421=CARTESIAN_POINT('Ctrl Pts',(-17.1654855522993,17.3122742668584,
-1.28932407812809E-15));
#118422=CARTESIAN_POINT('Ctrl Pts',(-17.2292149096655,17.2508596682763,
-5.87214431812852E-15));
#118423=CARTESIAN_POINT('Ctrl Pts',(-17.2958559710253,17.1929205201455,
-8.43769498715119E-15));
#118424=CARTESIAN_POINT('Ctrl Pts',(-17.3510488277484,17.1449346832427,
-1.05625121434475E-14));
#118425=CARTESIAN_POINT('Ctrl Pts',(-17.4082400420401,17.099332805993,-4.53394044041895E-15));
#118426=CARTESIAN_POINT('Ctrl Pts',(-17.467277750751,17.0562847197858,6.7168492989822E-15));
#118427=CARTESIAN_POINT('Ctrl Pts',(-17.4867746862249,17.042068284606,1.03075517856999E-14));
#118428=CARTESIAN_POINT('Ctrl Pts',(-17.5064731567169,17.0281304980274,
1.80459611682673E-14));
#118429=CARTESIAN_POINT('Ctrl Pts',(-17.5263681208433,17.0144778848536,
3.1641356201817E-15));
#118430=CARTESIAN_POINT('Ctrl Pts',(-17.5422931383847,17.0035495864712,
-8.70945017928273E-15));
#118431=CARTESIAN_POINT('Ctrl Pts',(-17.5583454202066,16.9928032530657,
3.52998690900286E-15));
#118432=CARTESIAN_POINT('Ctrl Pts',(-17.5745064361378,16.9822524120729,
5.10702591327572E-15));
#118433=CARTESIAN_POINT('Ctrl Pts',(-17.6490341987622,16.9335964008203,
1.25639560294472E-14));
#118434=CARTESIAN_POINT('Ctrl Pts',(-17.7259441000136,16.8890440749741,
4.67377112410806E-15));
#118435=CARTESIAN_POINT('Ctrl Pts',(-17.8049552753632,16.8488860377447,
8.13238365537927E-15));
#118436=CARTESIAN_POINT('Ctrl Pts',(-17.8827964927913,16.8093226406223,
1.16249942035744E-14));
#118437=CARTESIAN_POINT('Ctrl Pts',(-17.9626778959223,16.774023635519,1.251775654464E-14));
#118438=CARTESIAN_POINT('Ctrl Pts',(-18.0443633532837,16.7433042678249,
-2.16493489801906E-14));
#118439=CARTESIAN_POINT('Ctrl Pts',(-18.0530581203136,16.7400344355435,
-2.53480777024185E-14));
#118440=CARTESIAN_POINT('Ctrl Pts',(-18.0617733522417,16.7368165315127,
1.30580969649654E-14));
#118441=CARTESIAN_POINT('Ctrl Pts',(-18.0705086335888,16.7336504254972,
-1.0769163338864E-14));
#118442=CARTESIAN_POINT('Ctrl Pts',(-19.3965839091051,16.7348410960496,
-0.00189100554319391));
#118443=CARTESIAN_POINT('Ctrl Pts',(-20.2210098321597,16.9554454159071,
-0.044282941103672));
#118444=CARTESIAN_POINT('Ctrl Pts',(-21.6178061486211,18.2812774518108,
-0.129066812224628));
#118445=CARTESIAN_POINT('Ctrl Pts',(-21.0759342831862,21.1381886893359,
-0.256242618906062));
#118446=CARTESIAN_POINT('Ctrl Pts',(-18.3814920744256,22.2205668231227,
-0.383418425587496));
#118447=CARTESIAN_POINT('Ctrl Pts',(-16.012474196746,20.5450470987711,-0.510594232268932));
#118448=CARTESIAN_POINT('Ctrl Pts',(-16.139244329641,17.6439817266502,-0.637770038950364));
#118449=CARTESIAN_POINT('Ctrl Pts',(-18.647082433769,16.1814077892925,-0.764945845631801));
#118450=CARTESIAN_POINT('Ctrl Pts',(-21.2343814795738,17.4978560455519,
-0.892121652313232));
#118451=CARTESIAN_POINT('Ctrl Pts',(-21.5278812831845,20.386236189992,-1.01929745899467));
#118452=CARTESIAN_POINT('Ctrl Pts',(-19.2580928727389,22.1962914237501,
-1.14647326567611));
#118453=CARTESIAN_POINT('Ctrl Pts',(-16.5075209839662,21.267588636987,-1.27364907235753));
#118454=CARTESIAN_POINT('Ctrl Pts',(-15.7995850569884,18.4520614691495,
-1.40082487903898));
#118455=CARTESIAN_POINT('Ctrl Pts',(-17.7838032676266,16.3328298801955,
-1.52800068572041));
#118456=CARTESIAN_POINT('Ctrl Pts',(-20.6397625254543,16.8541321316718,
-1.65517649240185));
#118457=CARTESIAN_POINT('Ctrl Pts',(-21.747305794399,19.5377188342137,-1.78235229908328));
#118458=CARTESIAN_POINT('Ctrl Pts',(-20.0903265483327,21.9215589674176,
-1.90952810576472));
#118459=CARTESIAN_POINT('Ctrl Pts',(-17.1890026429968,21.8186306868887,
-2.03670391244613));
#118460=CARTESIAN_POINT('Ctrl Pts',(-15.7051175219999,19.3233624748623,
-2.16387971912758));
#118461=CARTESIAN_POINT('Ctrl Pts',(-17.0000442871287,16.7250089900212,
-2.29105552580901));
#118462=CARTESIAN_POINT('Ctrl Pts',(-19.8857676903764,16.4073977907608,
-2.41823133249045));
#118463=CARTESIAN_POINT('Ctrl Pts',(-21.714815780002,18.6619176945194,-2.54540713917187));
#118464=CARTESIAN_POINT('Ctrl Pts',(-20.8091503729495,21.4201864884025,
-2.67258294585332));
#118465=CARTESIAN_POINT('Ctrl Pts',(-17.9996633120291,22.1516638202427,
-2.79975875253474));
#118466=CARTESIAN_POINT('Ctrl Pts',(-15.8638845764857,20.1852646030015,
-2.92693455921619));
#118467=CARTESIAN_POINT('Ctrl Pts',(-16.3612586065906,17.3250380885132,
-3.05411036589761));
#118468=CARTESIAN_POINT('Ctrl Pts',(-19.0354755941188,16.1950645685336,
-3.18128617257904));
#118469=CARTESIAN_POINT('Ctrl Pts',(-21.4331074368131,17.832024618564,-3.30846197926049));
#118470=CARTESIAN_POINT('Ctrl Pts',(-21.3544757311695,20.7341089913131,
-3.43563778594193));
#118471=CARTESIAN_POINT('Ctrl Pts',(-18.8717201875366,22.2388353997967,
-3.56281359262336));
#118472=CARTESIAN_POINT('Ctrl Pts',(-16.2626149195662,20.9657107573881,
-3.68998939930478));
#118473=CARTESIAN_POINT('Ctrl Pts',(-15.9208520715149,18.0827479048318,
-3.81716520598622));
#118474=CARTESIAN_POINT('Ctrl Pts',(-18.1599778441558,16.2348863223055,
-3.94434101266766));
#118475=CARTESIAN_POINT('Ctrl Pts',(-20.9257333169718,17.11742432065,-4.0715168193491));
#118476=CARTESIAN_POINT('Ctrl Pts',(-21.6807095057666,19.9206880628195,
-4.19869262603053));
#118477=CARTESIAN_POINT('Ctrl Pts',(-19.7322626164446,22.0728570555698,
-4.32586843271195));
#118478=CARTESIAN_POINT('Ctrl Pts',(-16.8679717356974,21.5994498267117,
-4.4530442393934));
#118479=CARTESIAN_POINT('Ctrl Pts',(-15.7156459686732,18.934788125763,-4.58022004607482));
#118480=CARTESIAN_POINT('Ctrl Pts',(-17.3324726852114,16.5235336757831,
-4.70739585275626));
#118481=CARTESIAN_POINT('Ctrl Pts',(-20.2351137244727,16.5778627753009,
-4.8345716594377));
#118482=CARTESIAN_POINT('Ctrl Pts',(-21.7605760911555,19.0479318475521,
-4.96174746611912));
#118483=CARTESIAN_POINT('Ctrl Pts',(-20.5093427447009,21.6676058285233,
-5.08892327280056));
#118484=CARTESIAN_POINT('Ctrl Pts',(-17.6293426201811,22.033496435978,-5.216099079482));
#118485=CARTESIAN_POINT('Ctrl Pts',(-15.7627970788757,19.8099217473088,
-5.34327488616344));
#118486=CARTESIAN_POINT('Ctrl Pts',(-16.6221458040505,17.0368735287597,
-5.47045069284487));
#118487=CARTESIAN_POINT('Ctrl Pts',(-19.4189896775549,16.2584514060663,
-5.59762649952629));
#118488=CARTESIAN_POINT('Ctrl Pts',(-21.5873980371568,18.1888093624738,
-5.72480230620775));
#118489=CARTESIAN_POINT('Ctrl Pts',(-21.1379907995229,21.0569637845056,
-5.85197811288917));
#118490=CARTESIAN_POINT('Ctrl Pts',(-18.4830712118232,22.2315610076874,
-5.9791539195706));
#118491=CARTESIAN_POINT('Ctrl Pts',(-16.0583632128787,20.6349809834757,
-6.10632972625204));
#118492=CARTESIAN_POINT('Ctrl Pts',(-16.0883858973698,17.7319867891525,
-6.23350553293348));
#118493=CARTESIAN_POINT('Ctrl Pts',(-18.545595315694,16.1858954178693,-6.36068133961492));
#118494=CARTESIAN_POINT('Ctrl Pts',(-21.1756543381554,17.4151497415253,
-6.48785714629634));
#118495=CARTESIAN_POINT('Ctrl Pts',(-21.5656470515186,20.2919852142942,
-6.61503295297777));
#118496=CARTESIAN_POINT('Ctrl Pts',(-19.3577793469507,22.1770838464573,
-6.74220875965922));
#118497=CARTESIAN_POINT('Ctrl Pts',(-16.577632807668,21.3409846454216,-6.86938456634065));
#118498=CARTESIAN_POINT('Ctrl Pts',(-15.7758193281077,18.5507567339681,
-6.99656037302208));
#118499=CARTESIAN_POINT('Ctrl Pts',(-17.6879530096092,16.3662610397804,
-7.12373617970353));
#118500=CARTESIAN_POINT('Ctrl Pts',(-20.5597698797958,16.7916367771814,
-7.25091198638494));
#118501=CARTESIAN_POINT('Ctrl Pts',(-21.7565562053286,19.4366281089017,
-7.3780877930664));
#118502=CARTESIAN_POINT('Ctrl Pts',(-20.1803348134679,21.8746196547645,
-7.50526359974781));
#118503=CARTESIAN_POINT('Ctrl Pts',(-17.277190999913,21.8689054902615,-7.63243940642925));
#118504=CARTESIAN_POINT('Ctrl Pts',(-15.710579024174,19.4247280066634,-7.75961521311068));
#118505=CARTESIAN_POINT('Ctrl Pts',(-16.917768139086,16.7844683424076,-7.88679101979213));
#118506=CARTESIAN_POINT('Ctrl Pts',(-19.7912372583239,16.3704008664529,
-8.01396682647355));
#118507=CARTESIAN_POINT('Ctrl Pts',(-21.6947568125944,18.5624067880616,
-8.14114263315499));
#118508=CARTESIAN_POINT('Ctrl Pts',(-20.8819657566022,21.3494567253891,
-8.26831843983642));
#118509=CARTESIAN_POINT('Ctrl Pts',(-18.0985494367176,22.1746053447652,
-8.39549424651787));
#118510=CARTESIAN_POINT('Ctrl Pts',(-15.8981195681347,20.2808300024119,
-8.52267005319928));
#118511=CARTESIAN_POINT('Ctrl Pts',(-16.2994339811977,17.4055520339842,
-8.64984585988073));
#118512=CARTESIAN_POINT('Ctrl Pts',(-18.9343116103032,16.1866605156374,
-8.77702166656217));
#118513=CARTESIAN_POINT('Ctrl Pts',(-21.385415769696,17.7424127625149,-8.9041974732436));
#118514=CARTESIAN_POINT('Ctrl Pts',(-21.404010525815,20.6455026489812,-9.03137327992503));
#118515=CARTESIAN_POINT('Ctrl Pts',(-18.9730363440416,22.2325253902829,
-9.15854908660645));
#118516=CARTESIAN_POINT('Ctrl Pts',(-16.3227611528787,21.0474861230161,
-9.28572489328791));
#118517=CARTESIAN_POINT('Ctrl Pts',(-15.8846479455884,18.1775848230658,
-9.41290069996933));
#118518=CARTESIAN_POINT('Ctrl Pts',(-18.0606383974872,16.2557778069732,
-9.54007650665076));
#118519=CARTESIAN_POINT('Ctrl Pts',(-20.8543963261569,17.0452037312071,
-9.6672523133322));
#118520=CARTESIAN_POINT('Ctrl Pts',(-21.7028222322161,19.8216133075818,
-9.79442812001363));
#118521=CARTESIAN_POINT('Ctrl Pts',(-19.8275380061061,22.0378230731863,
-9.92160392669508));
#118522=CARTESIAN_POINT('Ctrl Pts',(-16.9490005320169,21.6605981215696,
-10.0487797333765));
#118523=CARTESIAN_POINT('Ctrl Pts',(-15.7080892802405,19.0360189326189,
-10.175955540058));
#118524=CARTESIAN_POINT('Ctrl Pts',(-17.2432633046432,16.5719740124406,
-10.3031313467394));
#118525=CARTESIAN_POINT('Ctrl Pts',(-20.1460957214815,16.5290716394223,
-10.4303071534208));
#118526=CARTESIAN_POINT('Ctrl Pts',(-21.7534179584053,18.9466720779869,
-10.5574829601022));
#118527=CARTESIAN_POINT('Ctrl Pts',(-20.5906116247063,21.6067769789573,
-10.6846587667837));
#118528=CARTESIAN_POINT('Ctrl Pts',(-17.7244793596526,22.0689052004239,
-10.8118345734651));
#118529=CARTESIAN_POINT('Ctrl Pts',(-15.7845196242002,19.9090827821031,
-10.9390103801465));
#118530=CARTESIAN_POINT('Ctrl Pts',(-16.5505250681459,17.1088127391066,
-11.066186186828));
#118531=CARTESIAN_POINT('Ctrl Pts',(-19.3197332403295,16.2371690315234,
-11.1933619935094));
#118532=CARTESIAN_POINT('Ctrl Pts',(-21.5515675192157,18.0938306607512,
-11.3205378001909));
#118533=CARTESIAN_POINT('Ctrl Pts',(-21.1984584771842,20.9754258193904,
-11.4477136068723));
#118534=CARTESIAN_POINT('Ctrl Pts',(-18.5843617438802,22.2382698013562,
-11.5748894135537));
#118535=CARTESIAN_POINT('Ctrl Pts',(-16.1075488229684,20.7237816341318,
-11.7020652202351));
#118536=CARTESIAN_POINT('Ctrl Pts',(-16.0403418410383,17.821410211409,-11.8292410269166));
#118537=CARTESIAN_POINT('Ctrl Pts',(-18.4443990326749,16.1939011720493,
-11.956416833598));
#118538=CARTESIAN_POINT('Ctrl Pts',(-21.1141471371691,17.3343930450618,
-12.0835926402795));
#118539=CARTESIAN_POINT('Ctrl Pts',(-21.6002579719026,20.1965553238665,
-12.2107684469609));
#118540=CARTESIAN_POINT('Ctrl Pts',(-19.4567550174485,22.1545317634858,
-12.3379442536423));
#118541=CARTESIAN_POINT('Ctrl Pts',(-16.650169193721,21.4120005062924,-12.4651200603238));
#118542=CARTESIAN_POINT('Ctrl Pts',(-15.7553687976281,18.6501878940739,
-12.5922958670052));
#118543=CARTESIAN_POINT('Ctrl Pts',(-17.593277655009,16.4028855811176,-12.7194716736866));
#118544=CARTESIAN_POINT('Ctrl Pts',(-20.4777284627055,16.7318539562487,
-12.8466474803681));
#118545=CARTESIAN_POINT('Ctrl Pts',(-21.7624166338639,19.3352849533645,
-12.9738232870495));
#118546=CARTESIAN_POINT('Ctrl Pts',(-20.268720508187,21.8246922197625,-13.1009990937309));
#118547=CARTESIAN_POINT('Ctrl Pts',(-17.3670135717459,21.9161990985631,
-13.2281749004124));
#118548=CARTESIAN_POINT('Ctrl Pts',(-15.7194318384815,19.5258537080241,
-13.3553507070938));
#118549=CARTESIAN_POINT('Ctrl Pts',(-16.8375292882087,16.846649582398,-13.4825265137753));
#118550=CARTESIAN_POINT('Ctrl Pts',(-19.6955209077569,16.3365902167848,
-13.6097023204567));
#118551=CARTESIAN_POINT('Ctrl Pts',(-21.6713767731562,18.4636234212799,
-13.7368781271381));
#118552=CARTESIAN_POINT('Ctrl Pts',(-20.9523717633484,21.2763282493288,
-13.8640539338195));
#118553=CARTESIAN_POINT('Ctrl Pts',(-18.1981483483483,22.1942225973466,
-13.991229740501));
#118554=CARTESIAN_POINT('Ctrl Pts',(-15.9355355650342,20.3751953719755,
-14.1184055471824));
#118555=CARTESIAN_POINT('Ctrl Pts',(-16.2403402085095,17.4880911509308,
-14.2455813538639));
#118556=CARTESIAN_POINT('Ctrl Pts',(-18.8329229366954,16.181648863124,-14.3727571605453));
#118557=CARTESIAN_POINT('Ctrl Pts',(-21.334750010313,17.6544482206642,-14.4999329672267));
#118558=CARTESIAN_POINT('Ctrl Pts',(-21.450550370219,20.555287225246,-14.6271087739081));
#118559=CARTESIAN_POINT('Ctrl Pts',(-19.0740843735804,22.2228261365397,
-14.7542845805896));
#118560=CARTESIAN_POINT('Ctrl Pts',(-16.3856120721985,21.1272015025705,
-14.881460387271));
#118561=CARTESIAN_POINT('Ctrl Pts',(-15.8516399371812,18.2735809228713,
-15.0086361939525));
#118562=CARTESIAN_POINT('Ctrl Pts',(-17.9620542603586,16.2799841636479,
-15.1358120006339));
#118563=CARTESIAN_POINT('Ctrl Pts',(-20.7806808873008,16.9754125149182,
-15.2629878073153));
#118564=CARTESIAN_POINT('Ctrl Pts',(-21.7216048314868,19.7218536275428,
-15.3901636139968));
#118565=CARTESIAN_POINT('Ctrl Pts',(-19.9215867744523,21.999618244049,-15.5173394206782));
#118566=CARTESIAN_POINT('Ctrl Pts',(-17.0320315618059,21.7189987028083,
-15.6445152273596));
#118567=CARTESIAN_POINT('Ctrl Pts',(-15.7039267551279,19.1374460156962,
-15.771691034041));
#118568=CARTESIAN_POINT('Ctrl Pts',(-17.1557260830642,16.6233745439076,
-15.8988668407225));
#118569=CARTESIAN_POINT('Ctrl Pts',(-20.0554937710623,16.483288821935,-16.0260426474039));
#118570=CARTESIAN_POINT('Ctrl Pts',(-21.7428729452643,18.8457088049877,
-16.1532184540854));
#118571=CARTESIAN_POINT('Ctrl Pts',(-20.669797943903,21.5432607869357,-16.2803942607668));
#118572=CARTESIAN_POINT('Ctrl Pts',(-17.8207484781814,22.1011082533001,
-16.4075700674482));
#118573=CARTESIAN_POINT('Ctrl Pts',(-15.8095506009463,20.0074607776102,
-16.5347458741296));
#118574=CARTESIAN_POINT('Ctrl Pts',(-16.4813535355424,17.1831099723939,
-16.6619216808111));
#118575=CARTESIAN_POINT('Ctrl Pts',(-19.2198197862706,16.2192224024562,
-16.7890974874925));
#118576=CARTESIAN_POINT('Ctrl Pts',(-21.5125765364721,18.0001050876052,
-16.916273294174));
#118577=CARTESIAN_POINT('Ctrl Pts',(-21.2561617723699,20.891908698262,-17.0434491008554));
#118578=CARTESIAN_POINT('Ctrl Pts',(-18.6858201251326,22.2415829072234,
-17.1706249075368));
#118579=CARTESIAN_POINT('Ctrl Pts',(-16.1596805227059,20.8108853979961,
-17.2978007142183));
#118580=CARTESIAN_POINT('Ctrl Pts',(-15.9953192604098,17.9123923361942,
-17.4249765208997));
#118581=CARTESIAN_POINT('Ctrl Pts',(-18.3435275949907,16.2052912052522,
-17.5521523275811));
#118582=CARTESIAN_POINT('Ctrl Pts',(-21.0499701257169,17.2557413381646,
-17.6793281342626));
#118583=CARTESIAN_POINT('Ctrl Pts',(-21.6316538114152,20.1000199362705,
-17.806503940944));
#118584=CARTESIAN_POINT('Ctrl Pts',(-19.5549199738189,22.1286779216513,
-17.9336797476255));
#118585=CARTESIAN_POINT('Ctrl Pts',(-16.7250430122834,21.4805475054267,
-18.0608555543069));
#118586=CARTESIAN_POINT('Ctrl Pts',(-15.7382593970452,18.7502481169883,
-18.1880313609883));
#118587=CARTESIAN_POINT('Ctrl Pts',(-17.4998818483857,16.4426599837058,
-18.3152071676697));
#118588=CARTESIAN_POINT('Ctrl Pts',(-20.3937311058227,16.6748519928531,
-18.4423829743512));
#118589=CARTESIAN_POINT('Ctrl Pts',(-21.7648800881945,19.2338023873838,
-18.5695587810326));
#118590=CARTESIAN_POINT('Ctrl Pts',(-20.355384707288,21.7718330069121,-18.6967345877141));
#118591=CARTESIAN_POINT('Ctrl Pts',(-17.458369491917,21.9604582855383,-18.8239103943955));
#118592=CARTESIAN_POINT('Ctrl Pts',(-15.7316660931769,19.6266262383536,
-18.9510862010769));
#118593=CARTESIAN_POINT('Ctrl Pts',(-16.7594177080439,16.911482913106,-19.0782620077583));
#118594=CARTESIAN_POINT('Ctrl Pts',(-19.5987260194682,16.3060037929748,
-19.2054378144398));
#118595=CARTESIAN_POINT('Ctrl Pts',(-21.6447018788134,18.3656783845019,
-19.3326136211212));
#118596=CARTESIAN_POINT('Ctrl Pts',(-21.0202894232019,21.2008830991641,
-19.4597894278026));
#118597=CARTESIAN_POINT('Ctrl Pts',(-18.298348324308,22.2104935619801,-19.5869652344841));
#118598=CARTESIAN_POINT('Ctrl Pts',(-15.9760905994637,20.468254879066,-19.7141410411655));
#118599=CARTESIAN_POINT('Ctrl Pts',(-16.1840435721468,17.5725628250383,
-19.841316847847));
#118600=CARTESIAN_POINT('Ctrl Pts',(-18.7314233036762,16.1800352894614,
-19.9684926545284));
#118601=CARTESIAN_POINT('Ctrl Pts',(-21.2811669856061,17.5682295538539,
-20.0956684612098));
#118602=CARTESIAN_POINT('Ctrl Pts',(-21.4940430697286,20.4635641243438,
-20.2228442678912));
#118603=CARTESIAN_POINT('Ctrl Pts',(-19.1747509132239,22.2097481144726,
-20.3500200745727));
#118604=CARTESIAN_POINT('Ctrl Pts',(-16.4510972110931,21.2047682572431,
-20.4771958812541));
#118605=CARTESIAN_POINT('Ctrl Pts',(-15.821865006984,18.370627026472,-20.6043716879356));
#118606=CARTESIAN_POINT('Ctrl Pts',(-17.8643361386242,16.3074811285329,
-20.731547494617));
#118607=CARTESIAN_POINT('Ctrl Pts',(-20.7046694479571,16.9081233905683,
-20.8587233012984));
#118608=CARTESIAN_POINT('Ctrl Pts',(-21.7370366957551,19.6215316486842,
-20.9858991079799));
#118609=CARTESIAN_POINT('Ctrl Pts',(-20.0143025394107,21.9582647545422,
-21.1130749146613));
#118610=CARTESIAN_POINT('Ctrl Pts',(-17.1169733995614,21.7746258892963,
-21.2402507213427));
#118611=CARTESIAN_POINT('Ctrl Pts',(-15.7031597664495,19.2388788584707,
-21.3674265280241));
#118612=CARTESIAN_POINT('Ctrl Pts',(-17.0699655633607,16.6778255053829,
-21.4946023347056));
#118613=CARTESIAN_POINT('Ctrl Pts',(-19.9633972500118,16.4402806602733,
-21.621778141387));
#118614=CARTESIAN_POINT('Ctrl Pts',(-21.7289765870023,18.7457048218335,
-21.7489539480685));
#118615=CARTESIAN_POINT('Ctrl Pts',(-20.7467662613402,21.4760665062299,
-21.8761297547499));
#118616=CARTESIAN_POINT('Ctrl Pts',(-17.9181406714293,22.1321446364483,
-22.0033055614313));
#118617=CARTESIAN_POINT('Ctrl Pts',(-15.8372831342433,20.1003769378317,
-22.1305000254672));
#118618=CARTESIAN_POINT('Ctrl Pts',(-16.2233209291158,18.2129921341989,
-22.2153025539425));
#118619=CARTESIAN_POINT('Ctrl Pts',(-16.7733106534418,17.5599162528134,
-22.2577131468574));
#118620=CARTESIAN_POINT('Ctrl Pts',(-19.3578031414673,16.879769673048,0.0847273919817681));
#118621=CARTESIAN_POINT('Ctrl Pts',(-20.133975749406,17.0874621114807,0.04233545642129));
#118622=CARTESIAN_POINT('Ctrl Pts',(-21.4490181436218,18.3356937357163,
-0.0424484146996662));
#118623=CARTESIAN_POINT('Ctrl Pts',(-20.9388618188364,21.0253911164874,
-0.1696242213811));
#118624=CARTESIAN_POINT('Ctrl Pts',(-18.402124220429,22.0444180968188,-0.296800028062535));
#118625=CARTESIAN_POINT('Ctrl Pts',(-16.1717639989072,20.466965862803,-0.423975834743969));
#118626=CARTESIAN_POINT('Ctrl Pts',(-16.291114327307,17.7356986710373,-0.551151641425403));
#118627=CARTESIAN_POINT('Ctrl Pts',(-18.6521696836906,16.3587285934148,
-0.678327448106839));
#118628=CARTESIAN_POINT('Ctrl Pts',(-21.0880351650422,17.5981256668252,
-0.80550325478827));
#118629=CARTESIAN_POINT('Ctrl Pts',(-21.3643565441105,20.3174500921447,
-0.932679061469707));
#118630=CARTESIAN_POINT('Ctrl Pts',(-19.2274179293257,22.0215635267321,
-1.05985486815114));
#118631=CARTESIAN_POINT('Ctrl Pts',(-16.6378358983264,21.1472173376516,
-1.18703067483258));
#118632=CARTESIAN_POINT('Ctrl Pts',(-15.9713351742103,18.4964818337432,
-1.31420648151401));
#118633=CARTESIAN_POINT('Ctrl Pts',(-17.8394178972337,16.5012880107125,
-1.44138228819545));
#118634=CARTESIAN_POINT('Ctrl Pts',(-20.5282190172933,16.9920786527069,
-1.56855809487688));
#118635=CARTESIAN_POINT('Ctrl Pts',(-21.5709382276219,19.5185961132746,
-1.69573390155831));
#118636=CARTESIAN_POINT('Ctrl Pts',(-20.0109413052122,21.7629110497128,
-1.82290970823975));
#118637=CARTESIAN_POINT('Ctrl Pts',(-17.2794307120758,21.6660071197238,
-1.95008551492118));
#118638=CARTESIAN_POINT('Ctrl Pts',(-15.8823967857546,19.316785944752,-2.07726132160262));
#118639=CARTESIAN_POINT('Ctrl Pts',(-17.101532012187,16.8705130362003,-2.20443712828405));
#118640=CARTESIAN_POINT('Ctrl Pts',(-19.8183551942992,16.5714914916967,
-2.33161293496548));
#118641=CARTESIAN_POINT('Ctrl Pts',(-21.5403498405985,18.6940552593023,
-2.45878874164692));
#118642=CARTESIAN_POINT('Ctrl Pts',(-20.6876926627317,21.2908836986755,
-2.58596454832835));
#118643=CARTESIAN_POINT('Ctrl Pts',(-18.0426437407308,21.9795479587692,
-2.71314035500979));
#118644=CARTESIAN_POINT('Ctrl Pts',(-16.0318712688937,20.128241290682,-2.84031616169122));
#118645=CARTESIAN_POINT('Ctrl Pts',(-16.5001341986149,17.4354226747645,
-2.96749196837266));
#118646=CARTESIAN_POINT('Ctrl Pts',(-19.0178303497907,16.3715860469025,
-3.09466777505409));
#118647=CARTESIAN_POINT('Ctrl Pts',(-21.275129772553,17.9127354887059,-3.22184358173553));
#118648=CARTESIAN_POINT('Ctrl Pts',(-21.2011003487691,20.6449620394061,
-3.34901938841696));
#118649=CARTESIAN_POINT('Ctrl Pts',(-18.8636594807816,22.0616174211049,
-3.4761951950984));
#118650=CARTESIAN_POINT('Ctrl Pts',(-16.4072640866091,20.8630082479868,
-3.60337100177983));
#118651=CARTESIAN_POINT('Ctrl Pts',(-16.0855044795293,18.1487840426529,
-3.73054680846126));
#118652=CARTESIAN_POINT('Ctrl Pts',(-18.1935751282717,16.4090770495669,
-3.8577226151427));
#118653=CARTESIAN_POINT('Ctrl Pts',(-20.7974520542944,17.2399604565832,
-3.98489842182413));
#118654=CARTESIAN_POINT('Ctrl Pts',(-21.50823979277,19.8791503081571,-4.11207422850556));
#118655=CARTESIAN_POINT('Ctrl Pts',(-19.6738347101252,21.9053537220903,
-4.239250035187));
#118656=CARTESIAN_POINT('Ctrl Pts',(-16.9771896136586,21.4596548264534,
-4.36642584186844));
#118657=CARTESIAN_POINT('Ctrl Pts',(-15.8923090067117,18.9509546948064,
-4.49360164854987));
#118658=CARTESIAN_POINT('Ctrl Pts',(-17.4145035108715,16.6808299904415,
-4.62077745523131));
#118659=CARTESIAN_POINT('Ctrl Pts',(-20.1472541466187,16.7319792297855,
-4.74795326191273));
#118660=CARTESIAN_POINT('Ctrl Pts',(-21.5834318192879,19.0574761604191,
-4.87512906859417));
#118661=CARTESIAN_POINT('Ctrl Pts',(-20.4054326534448,21.5238216851043,
-5.00230487527561));
#118662=CARTESIAN_POINT('Ctrl Pts',(-17.6939977688763,21.8682968636094,
-5.12948068195703));
#118663=CARTESIAN_POINT('Ctrl Pts',(-15.9367003815454,19.7748671001969,
-5.25665648863848));
#118664=CARTESIAN_POINT('Ctrl Pts',(-16.7457517741515,17.164124269893,-5.38383229531991));
#118665=CARTESIAN_POINT('Ctrl Pts',(-19.3788975093713,16.4312628785266,
-5.51100810200134));
#118666=CARTESIAN_POINT('Ctrl Pts',(-21.4203898065964,18.2486377661686,
-5.63818390868278));
#118667=CARTESIAN_POINT('Ctrl Pts',(-20.9972861924251,20.9489202724142,
-5.76535971536421));
#118668=CARTESIAN_POINT('Ctrl Pts',(-18.4977579720875,22.0547687962171,
-5.89253552204564));
#118669=CARTESIAN_POINT('Ctrl Pts',(-16.2149671495256,20.5516359536883,
-6.01971132872709));
#118670=CARTESIAN_POINT('Ctrl Pts',(-16.2432326184625,17.8185528329019,
-6.14688713540851));
#118671=CARTESIAN_POINT('Ctrl Pts',(-18.5566225655012,16.36295356291,-6.27406294208995));
#118672=CARTESIAN_POINT('Ctrl Pts',(-21.0327452994073,17.5202601292503,
-6.40123874877139));
#118673=CARTESIAN_POINT('Ctrl Pts',(-21.3999118973314,20.2287155878522,
-6.52841455545281));
#118674=CARTESIAN_POINT('Ctrl Pts',(-19.3212697946072,22.0034801611529,
-6.65559036213426));
#118675=CARTESIAN_POINT('Ctrl Pts',(-16.703844105405,21.2163175074616,-6.78276616881569));
#118676=CARTESIAN_POINT('Ctrl Pts',(-15.9489604438082,18.5894005047157,
-6.90994197549712));
#118677=CARTESIAN_POINT('Ctrl Pts',(-17.7491777159676,16.5327624580774,
-7.03711778217856));
#118678=CARTESIAN_POINT('Ctrl Pts',(-20.4529083087621,16.9332411259839,
-7.16429358885998));
#118679=CARTESIAN_POINT('Ctrl Pts',(-21.5796472157492,19.4234221871405,
-7.29146939554142));
#118680=CARTESIAN_POINT('Ctrl Pts',(-20.0956814230716,21.7187190760035,
-7.41864520222286));
#118681=CARTESIAN_POINT('Ctrl Pts',(-17.3624574402067,21.7133393592328,
-7.54582100890429));
#118682=CARTESIAN_POINT('Ctrl Pts',(-15.8875386284201,19.4122185930627,
-7.67299681558573));
#118683=CARTESIAN_POINT('Ctrl Pts',(-17.0240714537406,16.9264922567919,
-7.80017262226716));
#118684=CARTESIAN_POINT('Ctrl Pts',(-19.7293575901193,16.5366599823727,
-7.9273484289486));
#118685=CARTESIAN_POINT('Ctrl Pts',(-21.5214649164229,18.6003686858652,
-8.05452423563003));
#118686=CARTESIAN_POINT('Ctrl Pts',(-20.756246191493,21.2242937200225,-8.18170004231146));
#118687=CARTESIAN_POINT('Ctrl Pts',(-18.1357421006224,22.0011467251603,
-8.3088758489929));
#118688=CARTESIAN_POINT('Ctrl Pts',(-16.0641025003577,20.2182132859998,
-8.43605165567432));
#118689=CARTESIAN_POINT('Ctrl Pts',(-16.4419281434871,17.5112241716414,
-8.56322746235577));
#118690=CARTESIAN_POINT('Ctrl Pts',(-18.9225874529435,16.3636738798159,
-8.6904032690372));
#118691=CARTESIAN_POINT('Ctrl Pts',(-21.2302294793815,17.8283685782694,
-8.81757907571863));
#118692=CARTESIAN_POINT('Ctrl Pts',(-21.2477358919618,20.5615417903766,
-8.94475488240009));
#118693=CARTESIAN_POINT('Ctrl Pts',(-18.9590456437123,22.0556767338902,
-9.07193068908149));
#118694=CARTESIAN_POINT('Ctrl Pts',(-16.4638899852646,20.9399973346102,
-9.19910649576295));
#118695=CARTESIAN_POINT('Ctrl Pts',(-16.0514193664187,18.2380701945025,
-9.32628230244436));
#118696=CARTESIAN_POINT('Ctrl Pts',(-18.1000499791517,16.4287457641048,
-9.45345810912581));
#118697=CARTESIAN_POINT('Ctrl Pts',(-20.7302903886372,17.1719669089676,
-9.58063391580724));
#118698=CARTESIAN_POINT('Ctrl Pts',(-21.5290582703031,19.7858743581861,
-9.70780972248867));
#118699=CARTESIAN_POINT('Ctrl Pts',(-19.7635336698473,21.8723702644956,
-9.83498552917011));
#118700=CARTESIAN_POINT('Ctrl Pts',(-17.0534758273726,21.5172241363981,
-9.96216133585154));
#118701=CARTESIAN_POINT('Ctrl Pts',(-15.88519460819,19.0462605035686,-10.089337142533));
#118702=CARTESIAN_POINT('Ctrl Pts',(-17.3305155191891,16.7264351338286,
-10.2165129492144));
#118703=CARTESIAN_POINT('Ctrl Pts',(-20.0634463312613,16.6860438193137,
-10.3436887558959));
#118704=CARTESIAN_POINT('Ctrl Pts',(-21.5766926491464,18.9621430841235,
-10.4708645625773));
#118705=CARTESIAN_POINT('Ctrl Pts',(-20.4819448988438,21.466553123448,-10.5980403692588));
#118706=CARTESIAN_POINT('Ctrl Pts',(-17.7835661935479,21.9016331674242,
-10.7252161759402));
#118707=CARTESIAN_POINT('Ctrl Pts',(-15.9571515150968,19.8682242798172,
-10.8523919826216));
#118708=CARTESIAN_POINT('Ctrl Pts',(-16.6783229708898,17.2318529074172,
-10.9795677893031));
#118709=CARTESIAN_POINT('Ctrl Pts',(-19.2854505111856,16.4112261527396,
-11.1067435959845));
#118710=CARTESIAN_POINT('Ctrl Pts',(-21.3866564343474,18.1592181293605,
-11.2339194026659));
#118711=CARTESIAN_POINT('Ctrl Pts',(-21.0542147214219,20.8721546913479,
-11.3610952093473));
#118712=CARTESIAN_POINT('Ctrl Pts',(-18.5931200103587,22.0610849269117,
-11.4882710160288));
#118713=CARTESIAN_POINT('Ctrl Pts',(-16.261273945793,20.6352391382547,-11.6154468227102));
#118714=CARTESIAN_POINT('Ctrl Pts',(-16.1980005612746,17.9027423384994,
-11.7426226293916));
#118715=CARTESIAN_POINT('Ctrl Pts',(-18.4613492599099,16.3704907435428,
-11.8697984360731));
#118716=CARTESIAN_POINT('Ctrl Pts',(-20.9748380899644,17.4442300894981,
-11.9969742427545));
#118717=CARTESIAN_POINT('Ctrl Pts',(-21.4324970545739,20.138871170231,-12.124150049436));
#118718=CARTESIAN_POINT('Ctrl Pts',(-19.4144524592281,21.9822480424568,
-12.2513258561174));
#118719=CARTESIAN_POINT('Ctrl Pts',(-16.7721349661832,21.2831768387803,
-12.3785016627988));
#118720=CARTESIAN_POINT('Ctrl Pts',(-15.9297068745883,18.6830119993224,
-12.5056774694802));
#118721=CARTESIAN_POINT('Ctrl Pts',(-17.6600436714977,16.5672433798551,
-12.6328532761617));
#118722=CARTESIAN_POINT('Ctrl Pts',(-20.3756687425606,16.8769573693289,
-12.7600290828431));
#118723=CARTESIAN_POINT('Ctrl Pts',(-21.5851646357777,19.3280106054199,
-12.8872048895246));
#118724=CARTESIAN_POINT('Ctrl Pts',(-20.1788939389038,21.6717138735354,
-13.014380696206));
#118725=CARTESIAN_POINT('Ctrl Pts',(-17.4470227333175,21.7578648918097,
-13.1415565028874));
#118726=CARTESIAN_POINT('Ctrl Pts',(-15.8958732910946,19.5074254481115,
-13.2687323095689));
#118727=CARTESIAN_POINT('Ctrl Pts',(-16.9485289502823,16.9850340540092,
-13.3959081162503));
#118728=CARTESIAN_POINT('Ctrl Pts',(-19.6392434787545,16.5048282563255,
-13.5230839229317));
#118729=CARTESIAN_POINT('Ctrl Pts',(-21.4994533012164,18.5073670695018,
-13.6502597296132));
#118730=CARTESIAN_POINT('Ctrl Pts',(-20.8225313632018,21.1554454240253,
-13.7774355362946));
#118731=CARTESIAN_POINT('Ctrl Pts',(-18.2295115283253,22.0196157878994,
-13.904611342976));
#118732=CARTESIAN_POINT('Ctrl Pts',(-16.0993285541244,20.3070554887315,
-14.0317871496575));
#118733=CARTESIAN_POINT('Ctrl Pts',(-16.3862931053621,17.5889323075283,
-14.1589629563389));
#118734=CARTESIAN_POINT('Ctrl Pts',(-18.8271330173065,16.3589555572926,
-14.2861387630203));
#118735=CARTESIAN_POINT('Ctrl Pts',(-21.1825291663591,17.745552565399,-14.4133145697018));
#118736=CARTESIAN_POINT('Ctrl Pts',(-21.2915517781366,20.476606638826,-14.5404903763832));
#118737=CARTESIAN_POINT('Ctrl Pts',(-19.0541793730395,22.0465451735372,
-14.6676661830647));
#118738=CARTESIAN_POINT('Ctrl Pts',(-16.5230622657518,21.0150470053099,
-14.7948419897461));
#118739=CARTESIAN_POINT('Ctrl Pts',(-16.0203433033647,18.328447681496,-14.9220177964275));
#118740=CARTESIAN_POINT('Ctrl Pts',(-18.0072359316107,16.4515353325348,
-15.0491936031089));
#118741=CARTESIAN_POINT('Ctrl Pts',(-20.6608894845385,17.1062605442799,
-15.1763694097904));
#118742=CARTESIAN_POINT('Ctrl Pts',(-21.5467415316516,19.6919535717847,
-15.3035452164718));
#118743=CARTESIAN_POINT('Ctrl Pts',(-19.8520778019026,21.8364015485223,
-15.4307210231533));
#118744=CARTESIAN_POINT('Ctrl Pts',(-17.1316470846427,21.5722065552882,
-15.5578968298347));
#118745=CARTESIAN_POINT('Ctrl Pts',(-15.8812757139849,19.1417511005842,
-15.6850726365161));
#118746=CARTESIAN_POINT('Ctrl Pts',(-17.2481018157082,16.7748272130226,
-15.8122484431975));
#118747=CARTESIAN_POINT('Ctrl Pts',(-19.9781472762768,16.6429406515769,
-15.939424249879));
#118748=CARTESIAN_POINT('Ctrl Pts',(-21.5667648313502,18.8670891505701,
-16.0666000565604));
#118749=CARTESIAN_POINT('Ctrl Pts',(-20.5564964748742,21.4067545084005,
-16.1937758632419));
#118750=CARTESIAN_POINT('Ctrl Pts',(-17.8742007195895,21.9319513886684,
-16.3209516699233));
#118751=CARTESIAN_POINT('Ctrl Pts',(-15.9807174389196,19.9608442511223,
-16.4481274766047));
#118752=CARTESIAN_POINT('Ctrl Pts',(-16.6132000200527,17.3018015537547,
-16.5753032832862));
#118753=CARTESIAN_POINT('Ctrl Pts',(-19.1913849510953,16.3943299325974,
-16.7024790899676));
#118754=CARTESIAN_POINT('Ctrl Pts',(-21.3499475780197,18.0709782760213,
-16.829654896649));
#118755=CARTESIAN_POINT('Ctrl Pts',(-21.1085406661289,20.7935257934676,
-16.9568307033305));
#118756=CARTESIAN_POINT('Ctrl Pts',(-18.6886400736801,22.0642041180355,
-17.0840065100119));
#118757=CARTESIAN_POINT('Ctrl Pts',(-16.3103543982751,20.7172447541254,
-17.2111823166934));
#118758=CARTESIAN_POINT('Ctrl Pts',(-16.1556131340415,17.9883993163983,
-17.3383581233747));
#118759=CARTESIAN_POINT('Ctrl Pts',(-18.3663817865876,16.381214122719,-17.4655339300562));
#118760=CARTESIAN_POINT('Ctrl Pts',(-20.9144173329799,17.3701818351261,
-17.5927097367376));
#118761=CARTESIAN_POINT('Ctrl Pts',(-21.4620553083253,20.0479859597428,
-17.7198855434191));
#118762=CARTESIAN_POINT('Ctrl Pts',(-19.5068718604908,21.9579074155056,
-17.8470613501005));
#118763=CARTESIAN_POINT('Ctrl Pts',(-16.8426264504933,21.347711809839,-17.9742371567819));
#118764=CARTESIAN_POINT('Ctrl Pts',(-15.9135988802868,18.7772157379466,
-18.1014129634634));
#118765=CARTESIAN_POINT('Ctrl Pts',(-17.5721142835804,16.6046898027813,
-18.2285887701448));
#118766=CARTESIAN_POINT('Ctrl Pts',(-20.2965877169299,16.8232917077465,
-18.3557645768262));
#118767=CARTESIAN_POINT('Ctrl Pts',(-21.5874839051248,19.2324677728927,
-18.4829403835077));
#118768=CARTESIAN_POINT('Ctrl Pts',(-20.2604857175586,21.6219484889878,
-18.6101161901891));
#118769=CARTESIAN_POINT('Ctrl Pts',(-17.5330316285098,21.7995336065107,
-18.7372919968706));
#118770=CARTESIAN_POINT('Ctrl Pts',(-15.9073914798215,19.6022998030865,
-18.864467803552));
#118771=CARTESIAN_POINT('Ctrl Pts',(-16.874989209244,17.0460727161496,-18.9916436102334));
#118772=CARTESIAN_POINT('Ctrl Pts',(-19.5481139560441,16.4760320435035,
-19.1188194169148));
#118773=CARTESIAN_POINT('Ctrl Pts',(-21.4743396776274,18.4151547160267,
-19.2459952235963));
#118774=CARTESIAN_POINT('Ctrl Pts',(-20.8864738299528,21.08441604792,-19.3731710302777));
#118775=CARTESIAN_POINT('Ctrl Pts',(-18.3238468403057,22.0349344195679,
-19.5003468369591));
#118776=CARTESIAN_POINT('Ctrl Pts',(-16.1375099188267,20.3946682605915,
-19.6275226436406));
#118777=CARTESIAN_POINT('Ctrl Pts',(-16.3332914883073,17.6684598887888,
-19.754698450322));
#118778=CARTESIAN_POINT('Ctrl Pts',(-18.7315741166677,16.3574364254427,
-19.8818742570035));
#118779=CARTESIAN_POINT('Ctrl Pts',(-21.1320823343698,17.6643802422104,
-20.0090500636849));
#118780=CARTESIAN_POINT('Ctrl Pts',(-21.3324988675726,20.390252053842,-20.1362258703664));
#118781=CARTESIAN_POINT('Ctrl Pts',(-19.1489539409205,22.0342326028009,
-20.2634016770477));
#118782=CARTESIAN_POINT('Ctrl Pts',(-16.5847145860095,21.0880738092713,
-20.3905774837292));
#118783=CARTESIAN_POINT('Ctrl Pts',(-15.9923110877633,18.4198137159881,
-20.5177532904106));
#118784=CARTESIAN_POINT('Ctrl Pts',(-17.9152372119337,16.4774229112103,
-20.6449290970921));
#118785=CARTESIAN_POINT('Ctrl Pts',(-20.5893269639303,17.0429098251043,
-20.7721049037735));
#118786=CARTESIAN_POINT('Ctrl Pts',(-21.5612701751591,19.5975033976856,
-20.8992807104549));
#118787=CARTESIAN_POINT('Ctrl Pts',(-19.9393669507179,21.7974684619948,
-21.0264565171363));
#118788=CARTESIAN_POINT('Ctrl Pts',(-17.2116173110634,21.6245779050981,
-21.1536323238178));
#118789=CARTESIAN_POINT('Ctrl Pts',(-15.8805536168431,19.2372471201844,
-21.2808081304992));
#118790=CARTESIAN_POINT('Ctrl Pts',(-17.1673608244619,16.8260911817933,
-21.4079839371807));
#118791=CARTESIAN_POINT('Ctrl Pts',(-19.8914411272743,16.6024497401849,
-21.535159743862));
#118792=CARTESIAN_POINT('Ctrl Pts',(-21.5536818213048,18.7729383600156,
-21.6623355505436));
#118793=CARTESIAN_POINT('Ctrl Pts',(-20.628959867889,21.3434930817089,-21.7895113572249));
#118794=CARTESIAN_POINT('Ctrl Pts',(-17.9658925872421,21.9611712248908,
-21.9166871639064));
#118795=CARTESIAN_POINT('Ctrl Pts',(-16.0068267982834,20.0483220661474,
-22.0438816279422));
#118796=CARTESIAN_POINT('Ctrl Pts',(-16.370269957493,18.2714051300663,-22.1286841564175));
#118797=CARTESIAN_POINT('Ctrl Pts',(-16.8880690061789,17.6565535153103,
-22.1710947493324));
#118798=CARTESIAN_POINT('Ctrl Pts',(-19.3190223738293,17.0246982500464,
0.17134578950673));
#118799=CARTESIAN_POINT('Ctrl Pts',(-20.0469416666524,17.2194788070544,
0.128953853946252));
#118800=CARTESIAN_POINT('Ctrl Pts',(-21.2802301386225,18.3901100196218,
0.0441699828252958));
#118801=CARTESIAN_POINT('Ctrl Pts',(-20.8017893544867,20.9125935436388,
-0.0830058238561385));
#118802=CARTESIAN_POINT('Ctrl Pts',(-18.4227563664326,21.868269370515,-0.210181630537573));
#118803=CARTESIAN_POINT('Ctrl Pts',(-16.3310538010686,20.388884626835,-0.337357437219007));
#118804=CARTESIAN_POINT('Ctrl Pts',(-16.4429843249731,17.8274156154244,
-0.464533243900441));
#118805=CARTESIAN_POINT('Ctrl Pts',(-18.6572569336122,16.5360493975372,
-0.591709050581877));
#118806=CARTESIAN_POINT('Ctrl Pts',(-20.9416888505105,17.6983952880986,
-0.718884857263309));
#118807=CARTESIAN_POINT('Ctrl Pts',(-21.2008318050364,20.2486639942973,
-0.846060663944745));
#118808=CARTESIAN_POINT('Ctrl Pts',(-19.1967429859123,21.846835629714,-0.973236470626179));
#118809=CARTESIAN_POINT('Ctrl Pts',(-16.7681508126867,21.0268460383161,
-1.10041227730761));
#118810=CARTESIAN_POINT('Ctrl Pts',(-16.1430852914322,18.540902198337,-1.22758808398905));
#118811=CARTESIAN_POINT('Ctrl Pts',(-17.8950325268407,16.6697461412296,
-1.35476389067048));
#118812=CARTESIAN_POINT('Ctrl Pts',(-20.4166755091321,17.130025173742,-1.48193969735192));
#118813=CARTESIAN_POINT('Ctrl Pts',(-21.3945706608446,19.4994733923354,
-1.60911550403335));
#118814=CARTESIAN_POINT('Ctrl Pts',(-19.9315560620918,21.6042631320078,
-1.73629131071478));
#118815=CARTESIAN_POINT('Ctrl Pts',(-17.3698587811547,21.5133835525588,
-1.86346711739622));
#118816=CARTESIAN_POINT('Ctrl Pts',(-16.0596760495093,19.3102094146417,
-1.99064292407765));
#118817=CARTESIAN_POINT('Ctrl Pts',(-17.2030197372453,17.0160170823794,
-2.11781873075909));
#118818=CARTESIAN_POINT('Ctrl Pts',(-19.750942698222,16.7355851926327,-2.24499453744052));
#118819=CARTESIAN_POINT('Ctrl Pts',(-21.365883901195,18.7261928240851,-2.37217034412196));
#118820=CARTESIAN_POINT('Ctrl Pts',(-20.5662349525139,21.1615809089484,
-2.49934615080339));
#118821=CARTESIAN_POINT('Ctrl Pts',(-18.0856241694325,21.8074320972958,
-2.62652195748482));
#118822=CARTESIAN_POINT('Ctrl Pts',(-16.1998579613017,20.0712179783623,
-2.75369776416626));
#118823=CARTESIAN_POINT('Ctrl Pts',(-16.6390097906391,17.5458072610157,
-2.8808735708477));
#118824=CARTESIAN_POINT('Ctrl Pts',(-19.0001851054626,16.5481075252713,
-3.00804937752912));
#118825=CARTESIAN_POINT('Ctrl Pts',(-21.1171521082928,17.9934463588478,
-3.13522518421057));
#118826=CARTESIAN_POINT('Ctrl Pts',(-21.0477249663689,20.5558150874991,
-3.26240099089199));
#118827=CARTESIAN_POINT('Ctrl Pts',(-18.8555987740266,21.8843994424129,
-3.38957679757343));
#118828=CARTESIAN_POINT('Ctrl Pts',(-16.5519132536521,20.7603057385855,
-3.51675260425486));
#118829=CARTESIAN_POINT('Ctrl Pts',(-16.2501568875435,18.214820180474,-3.64392841093631));
#118830=CARTESIAN_POINT('Ctrl Pts',(-18.2271724123875,16.5832677768282,
-3.77110421761772));
#118831=CARTESIAN_POINT('Ctrl Pts',(-20.6691707916169,17.3624965925164,
-3.89828002429917));
#118832=CARTESIAN_POINT('Ctrl Pts',(-21.3357700797732,19.8376125534949,
-4.0254558309806));
#118833=CARTESIAN_POINT('Ctrl Pts',(-19.6154068038058,21.7378503886108,
-4.15263163766203));
#118834=CARTESIAN_POINT('Ctrl Pts',(-17.0864074916199,21.3198598261951,
-4.27980744434348));
#118835=CARTESIAN_POINT('Ctrl Pts',(-16.06897204475,18.9671212638499,-4.4069832510249));
#118836=CARTESIAN_POINT('Ctrl Pts',(-17.4965343365317,16.8381263050999,
-4.53415905770634));
#118837=CARTESIAN_POINT('Ctrl Pts',(-20.0593945687647,16.8860956842701,
-4.66133486438777));
#118838=CARTESIAN_POINT('Ctrl Pts',(-21.4062875474204,19.0670204732863,
-4.7885106710692));
#118839=CARTESIAN_POINT('Ctrl Pts',(-20.3015225621888,21.3800375416853,
-4.91568647775065));
#118840=CARTESIAN_POINT('Ctrl Pts',(-17.7586529175715,21.7030972912407,
-5.04286228443207));
#118841=CARTESIAN_POINT('Ctrl Pts',(-16.1106036842152,19.7398124530851,
-5.17003809111352));
#118842=CARTESIAN_POINT('Ctrl Pts',(-16.8693577442526,17.2913750110263,
-5.29721389779494));
#118843=CARTESIAN_POINT('Ctrl Pts',(-19.3388053411876,16.604074350987,-5.42438970447638));
#118844=CARTESIAN_POINT('Ctrl Pts',(-21.253381576036,18.3084661698633,-5.55156551115781));
#118845=CARTESIAN_POINT('Ctrl Pts',(-20.8565815853272,20.8408767603229,
-5.67874131783925));
#118846=CARTESIAN_POINT('Ctrl Pts',(-18.5124447323517,21.877976584747,-5.80591712452068));
#118847=CARTESIAN_POINT('Ctrl Pts',(-16.3715710861727,20.468290923901,-5.93309293120211));
#118848=CARTESIAN_POINT('Ctrl Pts',(-16.3980793395551,17.9051188766514,
-6.06026873788356));
#118849=CARTESIAN_POINT('Ctrl Pts',(-18.5676498153085,16.5400117079507,
-6.18744454456498));
#118850=CARTESIAN_POINT('Ctrl Pts',(-20.8898362606593,17.6253705169753,
-6.31462035124643));
#118851=CARTESIAN_POINT('Ctrl Pts',(-21.2341767431441,20.1654459614101,
-6.44179615792784));
#118852=CARTESIAN_POINT('Ctrl Pts',(-19.2847602422637,21.8298764758485,
-6.56897196460929));
#118853=CARTESIAN_POINT('Ctrl Pts',(-16.8300554031422,21.0916503695018,
-6.69614777129072));
#118854=CARTESIAN_POINT('Ctrl Pts',(-16.1221015595086,18.6280442754634,
-6.82332357797216));
#118855=CARTESIAN_POINT('Ctrl Pts',(-17.8104024223259,16.6992638763745,
-6.95049938465359));
#118856=CARTESIAN_POINT('Ctrl Pts',(-20.3460467377283,17.0748454747864,
-7.07767519133502));
#118857=CARTESIAN_POINT('Ctrl Pts',(-21.4027382261697,19.4102162653792,
-7.20485099801646));
#118858=CARTESIAN_POINT('Ctrl Pts',(-20.0110280326754,21.5628184972425,
-7.33202680469789));
#118859=CARTESIAN_POINT('Ctrl Pts',(-17.4477238805002,21.5577732282041,
-7.45920261137933));
#118860=CARTESIAN_POINT('Ctrl Pts',(-16.0644982326662,19.3997091794621,
-7.58637841806076));
#118861=CARTESIAN_POINT('Ctrl Pts',(-17.1303747683952,17.0685161711762,
-7.7135542247422));
#118862=CARTESIAN_POINT('Ctrl Pts',(-19.6674779219145,16.7029190982927,
-7.84073003142363));
#118863=CARTESIAN_POINT('Ctrl Pts',(-21.3481730202512,18.6383305836686,
-7.96790583810506));
#118864=CARTESIAN_POINT('Ctrl Pts',(-20.6305266263839,21.0991307146561,
-8.0950816447865));
#118865=CARTESIAN_POINT('Ctrl Pts',(-18.1729347645271,21.8276881055553,
-8.22225745146793));
#118866=CARTESIAN_POINT('Ctrl Pts',(-16.2300854325808,20.1555965695878,
-8.34943325814937));
#118867=CARTESIAN_POINT('Ctrl Pts',(-16.5844223057765,17.6168963092987,
-8.4766090648308));
#118868=CARTESIAN_POINT('Ctrl Pts',(-18.9108632955837,16.5406872439944,
-8.60378487151224));
#118869=CARTESIAN_POINT('Ctrl Pts',(-21.075043189067,17.9143243940239,-8.73096067819366));
#118870=CARTESIAN_POINT('Ctrl Pts',(-21.0914612581086,20.4775809317719,
-8.85813648487511));
#118871=CARTESIAN_POINT('Ctrl Pts',(-18.945054943383,21.8788280774976,-8.98531229155654));
#118872=CARTESIAN_POINT('Ctrl Pts',(-16.6050188176507,20.8325085462043,
-9.11248809823798));
#118873=CARTESIAN_POINT('Ctrl Pts',(-16.218190787249,18.2985555659393,-9.23966390491941));
#118874=CARTESIAN_POINT('Ctrl Pts',(-18.1394615608164,16.6017137212363,
-9.36683971160084));
#118875=CARTESIAN_POINT('Ctrl Pts',(-20.6061844511175,17.2987300867281,
-9.49401551828229));
#118876=CARTESIAN_POINT('Ctrl Pts',(-21.3552943083903,19.7501354087903,
-9.62119132496371));
#118877=CARTESIAN_POINT('Ctrl Pts',(-19.6995293335885,21.7069174558048,
-9.74836713164515));
#118878=CARTESIAN_POINT('Ctrl Pts',(-17.1579511227282,21.3738501512268,
-9.87554293832658));
#118879=CARTESIAN_POINT('Ctrl Pts',(-16.0622999361394,19.0565020745182,
-10.002718745008));
#118880=CARTESIAN_POINT('Ctrl Pts',(-17.4177677337352,16.8808962552165,
-10.1298945516894));
#118881=CARTESIAN_POINT('Ctrl Pts',(-19.980796941041,16.8430159992049,-10.2570703583709));
#118882=CARTESIAN_POINT('Ctrl Pts',(-21.3999673398873,18.9776140902601,
-10.3842461650523));
#118883=CARTESIAN_POINT('Ctrl Pts',(-20.3732781729815,21.3263292679386,
-10.5114219717337));
#118884=CARTESIAN_POINT('Ctrl Pts',(-17.8426530274432,21.7343611344247,
-10.6385977784151));
#118885=CARTESIAN_POINT('Ctrl Pts',(-16.1297834059933,19.8273657775314,
-10.7657735850966));
#118886=CARTESIAN_POINT('Ctrl Pts',(-16.8061208736337,17.3548930757276,
-10.892949391778));
#118887=CARTESIAN_POINT('Ctrl Pts',(-19.2511677820415,16.5852832739556,
-11.0201251984594));
#118888=CARTESIAN_POINT('Ctrl Pts',(-21.221745349479,18.2246055979698,-11.1473010051409));
#118889=CARTESIAN_POINT('Ctrl Pts',(-20.9099709656597,20.7688835633054,
-11.2744768118223));
#118890=CARTESIAN_POINT('Ctrl Pts',(-18.6018782768372,21.8839000524673,
-11.4016526185037));
#118891=CARTESIAN_POINT('Ctrl Pts',(-16.4149990686176,20.5466966423776,
-11.5288284251852));
#118892=CARTESIAN_POINT('Ctrl Pts',(-16.3556592815108,17.9840744655897,
-11.6560042318666));
#118893=CARTESIAN_POINT('Ctrl Pts',(-18.4782994871448,16.5470803150364,
-11.783180038548));
#118894=CARTESIAN_POINT('Ctrl Pts',(-20.8355290427597,17.5540671339344,
-11.9103558452295));
#118895=CARTESIAN_POINT('Ctrl Pts',(-21.2647361372453,20.0811870165956,
-12.0375316519109));
#118896=CARTESIAN_POINT('Ctrl Pts',(-19.3721499010078,21.8099643214279,
-12.1647074585924));
#118897=CARTESIAN_POINT('Ctrl Pts',(-16.8941007386454,21.1543531712681,
-12.2918832652738));
#118898=CARTESIAN_POINT('Ctrl Pts',(-16.1040449515487,18.7158361045709,
-12.4190590719552));
#118899=CARTESIAN_POINT('Ctrl Pts',(-17.7268096879864,16.7316011785925,
-12.5462348786367));
#118900=CARTESIAN_POINT('Ctrl Pts',(-20.2736090224157,17.0220607824092,
-12.6734106853181));
#118901=CARTESIAN_POINT('Ctrl Pts',(-21.4079126376915,19.3207362574753,
-12.8005864919995));
#118902=CARTESIAN_POINT('Ctrl Pts',(-20.0890673696206,21.5187355273081,
-12.9277622986809));
#118903=CARTESIAN_POINT('Ctrl Pts',(-17.5270318948891,21.5995306850564,
-13.0549381053624));
#118904=CARTESIAN_POINT('Ctrl Pts',(-16.0723147437075,19.4889971881991,
-13.1821139120438));
#118905=CARTESIAN_POINT('Ctrl Pts',(-17.0595286123559,17.1234185256205,
-13.3092897187253));
#118906=CARTESIAN_POINT('Ctrl Pts',(-19.5829660497523,16.6730662958661,
-13.4364655254067));
#118907=CARTESIAN_POINT('Ctrl Pts',(-21.3275298292767,18.5511107177236,
-13.5636413320881));
#118908=CARTESIAN_POINT('Ctrl Pts',(-20.6926909630551,21.0345625987219,
-13.6908171387696));
#118909=CARTESIAN_POINT('Ctrl Pts',(-18.2608747083023,21.8450089784522,
-13.817992945451));
#118910=CARTESIAN_POINT('Ctrl Pts',(-16.2631215432146,20.2389156054877,
-13.9451687521324));
#118911=CARTESIAN_POINT('Ctrl Pts',(-16.5322460022147,17.6897734641258,
-14.0723445588139));
#118912=CARTESIAN_POINT('Ctrl Pts',(-18.8213430979177,16.5362622514614,
-14.1995203654953));
#118913=CARTESIAN_POINT('Ctrl Pts',(-21.0303083224052,17.8366569101336,
-14.3266961721767));
#118914=CARTESIAN_POINT('Ctrl Pts',(-21.1325531860542,20.3979260524059,
-14.4538719788582));
#118915=CARTESIAN_POINT('Ctrl Pts',(-19.0342743724987,21.8702642105349,
-14.5810477855396));
#118916=CARTESIAN_POINT('Ctrl Pts',(-16.6605124593049,20.9028925080494,
-14.708223592221));
#118917=CARTESIAN_POINT('Ctrl Pts',(-16.1890466695481,18.3833144401207,
-14.8353993989025));
#118918=CARTESIAN_POINT('Ctrl Pts',(-18.0524176028627,16.6230865014217,
-14.9625752055839));
#118919=CARTESIAN_POINT('Ctrl Pts',(-20.5410980817764,17.2371085736416,
-15.0897510122653));
#118920=CARTESIAN_POINT('Ctrl Pts',(-21.3718782318164,19.6620535160264,
-15.2169268189468));
#118921=CARTESIAN_POINT('Ctrl Pts',(-19.7825688293528,21.6731848529956,
-15.3441026256282));
#118922=CARTESIAN_POINT('Ctrl Pts',(-17.2312626074793,21.4254144077681,
-15.4712784323096));
#118923=CARTESIAN_POINT('Ctrl Pts',(-16.0586246728421,19.1460561854722,
-15.5984542389911));
#118924=CARTESIAN_POINT('Ctrl Pts',(-17.3404775483521,16.9262798821378,
-15.7256300456725));
#118925=CARTESIAN_POINT('Ctrl Pts',(-19.9008007814914,16.8025924812187,
-15.852805852354));
#118926=CARTESIAN_POINT('Ctrl Pts',(-21.3906567174362,18.8884694961524,
-15.9799816590354));
#118927=CARTESIAN_POINT('Ctrl Pts',(-20.4431950058454,21.2702482298655,
-16.1071574657168));
#118928=CARTESIAN_POINT('Ctrl Pts',(-17.9276529609976,21.7627945240366,
-16.2343332723983));
#118929=CARTESIAN_POINT('Ctrl Pts',(-16.1518842768929,19.9142277246345,
-16.3615090790797));
#118930=CARTESIAN_POINT('Ctrl Pts',(-16.7450465045628,17.4204931351153,
-16.4886848857611));
#118931=CARTESIAN_POINT('Ctrl Pts',(-19.1629501159199,16.5694374627385,
-16.6158606924426));
#118932=CARTESIAN_POINT('Ctrl Pts',(-21.1873186195673,18.1418514644375,
-16.743036499124));
#118933=CARTESIAN_POINT('Ctrl Pts',(-20.960919559888,20.6951428886731,-16.8702123058054));
#118934=CARTESIAN_POINT('Ctrl Pts',(-18.6914600222275,21.8868253288476,
-16.9973881124868));
#118935=CARTESIAN_POINT('Ctrl Pts',(-16.4610282738444,20.6236041102547,
-17.1245639191683));
#118936=CARTESIAN_POINT('Ctrl Pts',(-16.3159070076732,18.0644062966023,
-17.2517397258497));
#118937=CARTESIAN_POINT('Ctrl Pts',(-18.3892359781844,16.5571370401859,
-17.3789155325312));
#118938=CARTESIAN_POINT('Ctrl Pts',(-20.7788645402429,17.4846223320876,
-17.5060913392126));
#118939=CARTESIAN_POINT('Ctrl Pts',(-21.2924568052356,19.9959519832151,
-17.633267145894));
#118940=CARTESIAN_POINT('Ctrl Pts',(-19.4588237471628,21.78713690936,-17.7604429525755));
#118941=CARTESIAN_POINT('Ctrl Pts',(-16.9602098887033,21.2148761142513,
-17.8876187592569));
#118942=CARTESIAN_POINT('Ctrl Pts',(-16.0889383635284,18.8041833589049,
-18.0147945659385));
#118943=CARTESIAN_POINT('Ctrl Pts',(-17.6443467187751,16.7667196218568,
-18.1419703726198));
#118944=CARTESIAN_POINT('Ctrl Pts',(-20.199444328037,16.97173142264,-18.2691461793012));
#118945=CARTESIAN_POINT('Ctrl Pts',(-21.410087722055,19.2311331584014,-18.3963219859826));
#118946=CARTESIAN_POINT('Ctrl Pts',(-20.1655867278293,21.4720639710636,
-18.5234977926641));
#118947=CARTESIAN_POINT('Ctrl Pts',(-17.6076937651026,21.638608927483,-18.6506735993455));
#118948=CARTESIAN_POINT('Ctrl Pts',(-16.083116866466,19.5779733678196,-18.777849406027));
#118949=CARTESIAN_POINT('Ctrl Pts',(-16.9905607104441,17.1806625191931,
-18.9050252127085));
#118950=CARTESIAN_POINT('Ctrl Pts',(-19.4975018926199,16.6460602940324,
-19.0322010193898));
#118951=CARTESIAN_POINT('Ctrl Pts',(-21.3039774764415,18.4646310475516,
-19.1593768260712));
#118952=CARTESIAN_POINT('Ctrl Pts',(-20.7526582367037,20.9679489966759,
-19.2865526327527));
#118953=CARTESIAN_POINT('Ctrl Pts',(-18.3493453563032,21.8593752771558,
-19.4137284394341));
#118954=CARTESIAN_POINT('Ctrl Pts',(-16.2989292381897,20.3210816421169,
-19.5409042461156));
#118955=CARTESIAN_POINT('Ctrl Pts',(-16.4825394044677,17.7643569525393,
-19.668080052797));
#118956=CARTESIAN_POINT('Ctrl Pts',(-18.7317249296591,16.5348375614239,
-19.7952558594784));
#118957=CARTESIAN_POINT('Ctrl Pts',(-20.9829976831335,17.760530930567,-19.9224316661598));
#118958=CARTESIAN_POINT('Ctrl Pts',(-21.1709546654166,20.31693998334,-20.0496074728413));
#118959=CARTESIAN_POINT('Ctrl Pts',(-19.1231569686169,21.8587170911293,
-20.1767832795227));
#118960=CARTESIAN_POINT('Ctrl Pts',(-16.7183319609261,20.9713793612995,
-20.3039590862042));
#118961=CARTESIAN_POINT('Ctrl Pts',(-16.1627571685425,18.4690004055044,
-20.4311348928856));
#118962=CARTESIAN_POINT('Ctrl Pts',(-17.9661382852434,16.6473646938876,
-20.558310699567));
#118963=CARTESIAN_POINT('Ctrl Pts',(-20.4739844799035,17.1776962596402,
-20.6854865062485));
#118964=CARTESIAN_POINT('Ctrl Pts',(-21.3855036545633,19.573475146687,-20.8126623129299));
#118965=CARTESIAN_POINT('Ctrl Pts',(-19.8644313620253,21.6366721694472,
-20.9398381196113));
#118966=CARTESIAN_POINT('Ctrl Pts',(-17.3062612225653,21.4745299209001,
-21.0670139262928));
#118967=CARTESIAN_POINT('Ctrl Pts',(-16.0579474672366,19.2356153818981,
-21.1941897329742));
#118968=CARTESIAN_POINT('Ctrl Pts',(-17.2647560855632,16.9743568582036,
-21.3213655396557));
#118969=CARTESIAN_POINT('Ctrl Pts',(-19.8194850045369,16.7646188200965,
-21.448541346337));
#118970=CARTESIAN_POINT('Ctrl Pts',(-21.3783870556072,18.8001718981978,
-21.5757171530185));
#118971=CARTESIAN_POINT('Ctrl Pts',(-20.5111534744378,21.210919657188,-21.7028929596999));
#118972=CARTESIAN_POINT('Ctrl Pts',(-18.013644503055,21.7901978133332,-21.8300687663814));
#118973=CARTESIAN_POINT('Ctrl Pts',(-16.1763704623236,19.996267194463,-21.9572632304172));
#118974=CARTESIAN_POINT('Ctrl Pts',(-16.5172189858702,18.3298181259339,
-22.0420657588926));
#118975=CARTESIAN_POINT('Ctrl Pts',(-17.0028273589161,17.7531907778071,
-22.0844763518074));
#118976=CARTESIAN_POINT('Ctrl Pts',(-19.2802416061914,17.1696268270448,
0.257964187031692));
#118977=CARTESIAN_POINT('Ctrl Pts',(-19.9599075838988,17.3514955026281,
0.215572251471214));
#118978=CARTESIAN_POINT('Ctrl Pts',(-21.1114421336233,18.4445263035272,
0.130788380350257));
#118979=CARTESIAN_POINT('Ctrl Pts',(-20.664716890137,20.7997959707902,0.00361257366882362));
#118980=CARTESIAN_POINT('Ctrl Pts',(-18.4433885124361,21.6921206442111,
-0.123563233012611));
#118981=CARTESIAN_POINT('Ctrl Pts',(-16.4903436032298,20.310803390867,-0.250739039694045));
#118982=CARTESIAN_POINT('Ctrl Pts',(-16.5948543226392,17.9191325598114,
-0.37791484637548));
#118983=CARTESIAN_POINT('Ctrl Pts',(-18.6623441835338,16.7133702016597,
-0.505090653056915));
#118984=CARTESIAN_POINT('Ctrl Pts',(-20.7953425359789,17.7986649093718,
-0.632266459738347));
#118985=CARTESIAN_POINT('Ctrl Pts',(-21.0373070659623,20.1798778964501,
-0.759442266419783));
#118986=CARTESIAN_POINT('Ctrl Pts',(-19.1660680424989,21.6721077326961,
-0.886618073101216));
#118987=CARTESIAN_POINT('Ctrl Pts',(-16.8984657270469,20.9064747389806,
-1.01379387978265));
#118988=CARTESIAN_POINT('Ctrl Pts',(-16.3148354086541,18.5853225629306,
-1.14096968646408));
#118989=CARTESIAN_POINT('Ctrl Pts',(-17.9506471564477,16.8382042717466,
-1.26814549314552));
#118990=CARTESIAN_POINT('Ctrl Pts',(-20.305132000971,17.2679716947772,-1.39532129982695));
#118991=CARTESIAN_POINT('Ctrl Pts',(-21.2182030940675,19.4803506713964,
-1.52249710650838));
#118992=CARTESIAN_POINT('Ctrl Pts',(-19.8521708189713,21.445615214303,-1.64967291318982));
#118993=CARTESIAN_POINT('Ctrl Pts',(-17.4602868502336,21.3607599853939,
-1.77684871987125));
#118994=CARTESIAN_POINT('Ctrl Pts',(-16.236955313264,19.3036328845313,-1.90402452655269));
#118995=CARTESIAN_POINT('Ctrl Pts',(-17.3045074623036,17.1615211285584,
-2.03120033323412));
#118996=CARTESIAN_POINT('Ctrl Pts',(-19.6835302021449,16.8996788935686,
-2.15837613991555));
#118997=CARTESIAN_POINT('Ctrl Pts',(-21.1914179617914,18.758330388868,-2.28555194659699));
#118998=CARTESIAN_POINT('Ctrl Pts',(-20.444777242296,21.0322781192214,-2.41272775327842));
#118999=CARTESIAN_POINT('Ctrl Pts',(-18.1286045981342,21.6353162358223,
-2.53990355995986));
#119000=CARTESIAN_POINT('Ctrl Pts',(-16.3678446537097,20.0141946660428,
-2.66707936664131));
#119001=CARTESIAN_POINT('Ctrl Pts',(-16.7778853826632,17.6561918472671,
-2.79425517332272));
#119002=CARTESIAN_POINT('Ctrl Pts',(-18.9825398611346,16.7246290036402,
-2.92143098000418));
#119003=CARTESIAN_POINT('Ctrl Pts',(-20.9591744440326,18.0741572289896,
-3.04860678668559));
#119004=CARTESIAN_POINT('Ctrl Pts',(-20.8943495839686,20.4666681355921,
-3.17578259336703));
#119005=CARTESIAN_POINT('Ctrl Pts',(-18.8475380672715,21.7071814637211,
-3.30295840004846));
#119006=CARTESIAN_POINT('Ctrl Pts',(-16.696562420695,20.6576032291843,-3.4301342067299));
#119007=CARTESIAN_POINT('Ctrl Pts',(-16.4148092955578,18.2808563182951,
-3.55731001341133));
#119008=CARTESIAN_POINT('Ctrl Pts',(-18.2607696965035,16.7574585040896,
-3.68448582009278));
#119009=CARTESIAN_POINT('Ctrl Pts',(-20.5408895289395,17.4850327284497,
-3.8116616267742));
#119010=CARTESIAN_POINT('Ctrl Pts',(-21.1633003667766,19.7960747988325,
-3.93883743345564));
#119011=CARTESIAN_POINT('Ctrl Pts',(-19.5569788974863,21.5703470551314,
-4.06601324013707));
#119012=CARTESIAN_POINT('Ctrl Pts',(-17.1956253695811,21.1800648259367,
-4.19318904681852));
#119013=CARTESIAN_POINT('Ctrl Pts',(-16.2456350827884,18.9832878328934,
-4.32036485349995));
#119014=CARTESIAN_POINT('Ctrl Pts',(-17.5785651621917,16.9954226197583,
-4.44754066018137));
#119015=CARTESIAN_POINT('Ctrl Pts',(-19.9715349909106,17.0402121387546,
-4.57471646686281));
#119016=CARTESIAN_POINT('Ctrl Pts',(-21.2291432755529,19.0765647861535,
-4.70189227354424));
#119017=CARTESIAN_POINT('Ctrl Pts',(-20.1976124709327,21.2362533982663,
-4.82906808022569));
#119018=CARTESIAN_POINT('Ctrl Pts',(-17.8233080662669,21.5378977188721,
-4.95624388690712));
#119019=CARTESIAN_POINT('Ctrl Pts',(-16.2845069868849,19.7047578059733,
-5.08341969358855));
#119020=CARTESIAN_POINT('Ctrl Pts',(-16.9929637143536,17.4186257521595,
-5.21059550026999));
#119021=CARTESIAN_POINT('Ctrl Pts',(-19.298713173004,16.7768858234474,-5.33777130695141));
#119022=CARTESIAN_POINT('Ctrl Pts',(-21.0863733454756,18.368294573558,-5.46494711363286));
#119023=CARTESIAN_POINT('Ctrl Pts',(-20.7158769782294,20.7328332482315,
-5.59212292031427));
#119024=CARTESIAN_POINT('Ctrl Pts',(-18.5271314926159,21.7011843732767,
-5.71929872699574));
#119025=CARTESIAN_POINT('Ctrl Pts',(-16.5281750228197,20.3849458941136,
-5.84647453367714));
#119026=CARTESIAN_POINT('Ctrl Pts',(-16.5529260606478,17.9916849204009,
-5.9736503403586));
#119027=CARTESIAN_POINT('Ctrl Pts',(-18.5786770651157,16.7170698529915,
-6.10082614704002));
#119028=CARTESIAN_POINT('Ctrl Pts',(-20.7469272219113,17.7304809047003,
-6.22800195372147));
#119029=CARTESIAN_POINT('Ctrl Pts',(-21.0684415889569,20.1021763349681,
-6.35517776040288));
#119030=CARTESIAN_POINT('Ctrl Pts',(-19.2482506899202,21.6562727905442,
-6.48235356708434));
#119031=CARTESIAN_POINT('Ctrl Pts',(-16.9562667008792,20.9669832315418,
-6.60952937376576));
#119032=CARTESIAN_POINT('Ctrl Pts',(-16.2952426752091,18.6666880462109,
-6.7367051804472));
#119033=CARTESIAN_POINT('Ctrl Pts',(-17.8716271286841,16.8657652946716,
-6.86388098712864));
#119034=CARTESIAN_POINT('Ctrl Pts',(-20.2391851666945,17.2164498235889,
-6.99105679381006));
#119035=CARTESIAN_POINT('Ctrl Pts',(-21.2258292365902,19.397010343618,-7.11823260049151));
#119036=CARTESIAN_POINT('Ctrl Pts',(-19.9263746422792,21.4069179184816,
-7.24540840717293));
#119037=CARTESIAN_POINT('Ctrl Pts',(-17.5329903207938,21.4022070971754,
-7.37258421385437));
#119038=CARTESIAN_POINT('Ctrl Pts',(-16.2414578369124,19.3871997658614,
-7.49976002053581));
#119039=CARTESIAN_POINT('Ctrl Pts',(-17.2366780830498,17.2105400855604,
-7.62693582721722));
#119040=CARTESIAN_POINT('Ctrl Pts',(-19.6055982537098,16.8691782142126,
-7.75411163389868));
#119041=CARTESIAN_POINT('Ctrl Pts',(-21.1748811240797,18.6762924814722,
-7.88128744058011));
#119042=CARTESIAN_POINT('Ctrl Pts',(-20.5048070612748,20.9739677092896,
-8.00846324726155));
#119043=CARTESIAN_POINT('Ctrl Pts',(-18.2101274284319,21.6542294859505,
-8.13563905394297));
#119044=CARTESIAN_POINT('Ctrl Pts',(-16.3960683648039,20.0929798531758,
-8.26281486062441));
#119045=CARTESIAN_POINT('Ctrl Pts',(-16.7269164680658,17.7225684469559,
-8.38999066730585));
#119046=CARTESIAN_POINT('Ctrl Pts',(-18.899139138224,16.717700608173,-8.51716647398728));
#119047=CARTESIAN_POINT('Ctrl Pts',(-20.9198568987526,18.0002802097783,
-8.64434228066872));
#119048=CARTESIAN_POINT('Ctrl Pts',(-20.9351866242553,20.3936200731671,
-8.77151808735015));
#119049=CARTESIAN_POINT('Ctrl Pts',(-18.9310642430538,21.7019794211049,
-8.89869389403158));
#119050=CARTESIAN_POINT('Ctrl Pts',(-16.7461476500366,20.7250197577984,
-9.02586970071301));
#119051=CARTESIAN_POINT('Ctrl Pts',(-16.3849622080794,18.3590409373758,
-9.15304550739446));
#119052=CARTESIAN_POINT('Ctrl Pts',(-18.1788731424809,16.774681678368,-9.28022131407588));
#119053=CARTESIAN_POINT('Ctrl Pts',(-20.4820785135977,17.4254932644886,
-9.40739712075733));
#119054=CARTESIAN_POINT('Ctrl Pts',(-21.1815303464774,19.7143964593946,
-9.53457292743875));
#119055=CARTESIAN_POINT('Ctrl Pts',(-19.6355249973296,21.5414646471141,
-9.66174873412019));
#119056=CARTESIAN_POINT('Ctrl Pts',(-17.2624264180838,21.2304761660553,
-9.78892454080163));
#119057=CARTESIAN_POINT('Ctrl Pts',(-16.2394052640888,19.0667436454676,
-9.91610034748306));
#119058=CARTESIAN_POINT('Ctrl Pts',(-17.5050199482811,17.0353573766044,
-10.0432761541645));
#119059=CARTESIAN_POINT('Ctrl Pts',(-19.8981475508207,16.9999881790961,
-10.1704519608459));
#119060=CARTESIAN_POINT('Ctrl Pts',(-21.2232420306283,18.9930850963969,
-10.2976277675273));
#119061=CARTESIAN_POINT('Ctrl Pts',(-20.264611447119,21.1861054124292,-10.4248035742088));
#119062=CARTESIAN_POINT('Ctrl Pts',(-17.9017398613385,21.5670891014251,
-10.5519793808902));
#119063=CARTESIAN_POINT('Ctrl Pts',(-16.30241529689,19.7865072752454,-10.6791551875716));
#119064=CARTESIAN_POINT('Ctrl Pts',(-16.9339187763774,17.477933244038,-10.8063309942531));
#119065=CARTESIAN_POINT('Ctrl Pts',(-19.2168850528976,16.7593403951717,
-10.9335068009345));
#119066=CARTESIAN_POINT('Ctrl Pts',(-21.0568342646105,18.289993066579,-11.0606826076159));
#119067=CARTESIAN_POINT('Ctrl Pts',(-20.7657272098974,20.6656124352628,
-11.1878584142974));
#119068=CARTESIAN_POINT('Ctrl Pts',(-18.6106365433157,21.7067151780229,
-11.3150342209788));
#119069=CARTESIAN_POINT('Ctrl Pts',(-16.5687241914422,20.4581541465005,
-11.4422100276602));
#119070=CARTESIAN_POINT('Ctrl Pts',(-16.5133180017472,18.0654065926801,
-11.5693858343417));
#119071=CARTESIAN_POINT('Ctrl Pts',(-18.4952497143798,16.7236698865299,
-11.6965616410231));
#119072=CARTESIAN_POINT('Ctrl Pts',(-20.696219995555,17.6639041783707,-11.8237374477046));
#119073=CARTESIAN_POINT('Ctrl Pts',(-21.0969752199166,20.0235028629602,
-11.950913254386));
#119074=CARTESIAN_POINT('Ctrl Pts',(-19.3298473427874,21.6376806003988,
-12.0780890610674));
#119075=CARTESIAN_POINT('Ctrl Pts',(-17.0160665111076,21.0255295037559,
-12.2052648677489));
#119076=CARTESIAN_POINT('Ctrl Pts',(-16.278383028509,18.7486602098194,-12.3324406744303));
#119077=CARTESIAN_POINT('Ctrl Pts',(-17.7935757044751,16.8959589773299,
-12.4596164811117));
#119078=CARTESIAN_POINT('Ctrl Pts',(-20.1715493022707,17.1671641954894,
-12.5867922877931));
#119079=CARTESIAN_POINT('Ctrl Pts',(-21.2306606396052,19.3134619095308,
-12.7139680944746));
#119080=CARTESIAN_POINT('Ctrl Pts',(-19.9992408003375,21.365757181081,-12.841143901156));
#119081=CARTESIAN_POINT('Ctrl Pts',(-17.6070410564606,21.4411964783031,
-12.9683197078375));
#119082=CARTESIAN_POINT('Ctrl Pts',(-16.2487561963206,19.4705689282866,
-13.0954955145189));
#119083=CARTESIAN_POINT('Ctrl Pts',(-17.1705282744295,17.2618029972318,
-13.2226713212003));
#119084=CARTESIAN_POINT('Ctrl Pts',(-19.52668862075,16.8413043354067,-13.3498471278818));
#119085=CARTESIAN_POINT('Ctrl Pts',(-21.1556063573368,18.5948543659455,
-13.4770229345632));
#119086=CARTESIAN_POINT('Ctrl Pts',(-20.5628505629085,20.9136797734184,
-13.6041987412446));
#119087=CARTESIAN_POINT('Ctrl Pts',(-18.2922378882792,21.670402169005,-13.7313745479261));
#119088=CARTESIAN_POINT('Ctrl Pts',(-16.4269145323048,20.1707757222437,
-13.8585503546075));
#119089=CARTESIAN_POINT('Ctrl Pts',(-16.6781988990673,17.7906146207234,
-13.9857261612889));
#119090=CARTESIAN_POINT('Ctrl Pts',(-18.8155531785289,16.7135689456302,
-14.1129019679704));
#119091=CARTESIAN_POINT('Ctrl Pts',(-20.8780874784513,17.9277612548684,
-14.2400777746518));
#119092=CARTESIAN_POINT('Ctrl Pts',(-20.9735545939718,20.3192454659859,
-14.3672535813332));
#119093=CARTESIAN_POINT('Ctrl Pts',(-19.0143693719578,21.6939832475324,
-14.4944293880147));
#119094=CARTESIAN_POINT('Ctrl Pts',(-16.7979626528582,20.7907380107889,
-14.6216051946961));
#119095=CARTESIAN_POINT('Ctrl Pts',(-16.3577500357315,18.4381811987453,
-14.7487810013775));
#119096=CARTESIAN_POINT('Ctrl Pts',(-18.0975992741149,16.7946376703086,
-14.875956808059));
#119097=CARTESIAN_POINT('Ctrl Pts',(-20.4213066790141,17.3679566030033,
-15.0031326147404));
#119098=CARTESIAN_POINT('Ctrl Pts',(-21.1970149319813,19.6321534602683,
-15.1303084214219));
#119099=CARTESIAN_POINT('Ctrl Pts',(-19.713059856803,21.5099681574688,-15.2574842281033));
#119100=CARTESIAN_POINT('Ctrl Pts',(-17.3308781303159,21.2786222602481,
-15.3846600347847));
#119101=CARTESIAN_POINT('Ctrl Pts',(-16.2359736316991,19.1503612703603,
-15.5118358414661));
#119102=CARTESIAN_POINT('Ctrl Pts',(-17.432853280996,17.0777325512529,-15.6390116481476));
#119103=CARTESIAN_POINT('Ctrl Pts',(-19.8234542867059,16.9622443108606,
-15.766187454829));
#119104=CARTESIAN_POINT('Ctrl Pts',(-21.2145486035221,18.9098498417347,
-15.8933632615105));
#119105=CARTESIAN_POINT('Ctrl Pts',(-20.3298935368166,21.1337419513304,
-16.0205390681919));
#119106=CARTESIAN_POINT('Ctrl Pts',(-17.9811052024058,21.5936376594049,
-16.1477148748733));
#119107=CARTESIAN_POINT('Ctrl Pts',(-16.3230511148663,19.8676111981466,
-16.2748906815548));
#119108=CARTESIAN_POINT('Ctrl Pts',(-16.8768929890729,17.5391847164761,
-16.4020664882362));
#119109=CARTESIAN_POINT('Ctrl Pts',(-19.1345152807445,16.7445449928796,
-16.5292422949176));
#119110=CARTESIAN_POINT('Ctrl Pts',(-21.0246896611148,18.2127246528537,
-16.656418101599));
#119111=CARTESIAN_POINT('Ctrl Pts',(-20.8132984536472,20.5967599838785,
-16.7835939082805));
#119112=CARTESIAN_POINT('Ctrl Pts',(-18.6942799707749,21.7094465396596,
-16.9107697149619));
#119113=CARTESIAN_POINT('Ctrl Pts',(-16.6117021494137,20.5299634663839,
-17.0379455216434));
#119114=CARTESIAN_POINT('Ctrl Pts',(-16.4762008813049,18.1404132768064,
-17.1651213283248));
#119115=CARTESIAN_POINT('Ctrl Pts',(-18.4120901697813,16.7330599576527,
-17.2922971350062));
#119116=CARTESIAN_POINT('Ctrl Pts',(-20.6433117475059,17.5990628290491,
-17.4194729416877));
#119117=CARTESIAN_POINT('Ctrl Pts',(-21.1228583021457,19.9439180066875,
-17.5466487483691));
#119118=CARTESIAN_POINT('Ctrl Pts',(-19.4107756338348,21.6163664032144,
-17.6738245550505));
#119119=CARTESIAN_POINT('Ctrl Pts',(-17.0777933269134,21.0820404186637,
-17.801000361732));
#119120=CARTESIAN_POINT('Ctrl Pts',(-16.2642778467699,18.8311509798632,
-17.9281761684134));
#119121=CARTESIAN_POINT('Ctrl Pts',(-17.7165791539697,16.9287494409323,
-18.0553519750948));
#119122=CARTESIAN_POINT('Ctrl Pts',(-20.1023009391443,17.1201711375333,
-18.1825277817763));
#119123=CARTESIAN_POINT('Ctrl Pts',(-21.2326915389853,19.2297985439103,
-18.3097035884577));
#119124=CARTESIAN_POINT('Ctrl Pts',(-20.0706877380999,21.3221794531393,
-18.4368793951392));
#119125=CARTESIAN_POINT('Ctrl Pts',(-17.6823559016955,21.4776842484555,
-18.5640552018205));
#119126=CARTESIAN_POINT('Ctrl Pts',(-16.2588422531106,19.5536469325526,
-18.691231008502));
#119127=CARTESIAN_POINT('Ctrl Pts',(-17.1061322116441,17.3152523222366,
-18.8184068151834));
#119128=CARTESIAN_POINT('Ctrl Pts',(-19.4468898291958,16.8160885445611,
-18.9455826218649));
#119129=CARTESIAN_POINT('Ctrl Pts',(-21.1336152752557,18.5141073790766,
-19.0727584285463));
#119130=CARTESIAN_POINT('Ctrl Pts',(-20.6188426434545,20.8514819454316,
-19.1999342352277));
#119131=CARTESIAN_POINT('Ctrl Pts',(-18.3748438723008,21.6838161347437,
-19.3271100419092));
#119132=CARTESIAN_POINT('Ctrl Pts',(-16.4603485575527,20.2474950236424,
-19.4542858485906));
#119133=CARTESIAN_POINT('Ctrl Pts',(-16.6317873206282,17.8602540162898,
-19.5814616552721));
#119134=CARTESIAN_POINT('Ctrl Pts',(-18.7318757426506,16.712238697405,-19.7086374619535));
#119135=CARTESIAN_POINT('Ctrl Pts',(-20.833913031897,17.8566816189236,-19.8358132686349));
#119136=CARTESIAN_POINT('Ctrl Pts',(-21.0094104632606,20.243627912838,-19.9629890753163));
#119137=CARTESIAN_POINT('Ctrl Pts',(-19.0973599963134,21.6832015794576,
-20.0901648819978));
#119138=CARTESIAN_POINT('Ctrl Pts',(-16.8519493358426,20.8546849133278,
-20.2173406886792));
#119139=CARTESIAN_POINT('Ctrl Pts',(-16.3332032493219,18.5181870950206,
-20.3445164953606));
#119140=CARTESIAN_POINT('Ctrl Pts',(-18.0170393585529,16.817306476565,-20.4716923020421));
#119141=CARTESIAN_POINT('Ctrl Pts',(-20.3586419958767,17.3124826941761,
-20.5988681087235));
#119142=CARTESIAN_POINT('Ctrl Pts',(-21.2097371339674,19.5494468956883,
-20.726043915405));
#119143=CARTESIAN_POINT('Ctrl Pts',(-19.7894957733326,21.4758758768998,
-20.8532197220864));
#119144=CARTESIAN_POINT('Ctrl Pts',(-17.4009051340672,21.3244819367018,
-20.9803955287679));
#119145=CARTESIAN_POINT('Ctrl Pts',(-16.2353413176302,19.2339836436119,
-21.1075713354492));
#119146=CARTESIAN_POINT('Ctrl Pts',(-17.3621513466646,17.1226225346138,
-21.2347471421307));
#119147=CARTESIAN_POINT('Ctrl Pts',(-19.7475288817995,16.9267879000082,
-21.3619229488121));
#119148=CARTESIAN_POINT('Ctrl Pts',(-21.2030922899096,18.82740543638,-21.4890987554935));
#119149=CARTESIAN_POINT('Ctrl Pts',(-20.3933470809866,21.078346232667,-21.616274562175));
#119150=CARTESIAN_POINT('Ctrl Pts',(-18.0613964188678,21.6192244017756,
-21.7434503688564));
#119151=CARTESIAN_POINT('Ctrl Pts',(-16.3459141263638,19.9442123227787,
-21.8706448328923));
#119152=CARTESIAN_POINT('Ctrl Pts',(-16.6641680142473,18.3882311218014,
-21.9554473613676));
#119153=CARTESIAN_POINT('Ctrl Pts',(-17.1175857116532,17.849828040304,-21.9978579542825));
#119154=CARTESIAN_POINT('Ctrl Pts',(-19.3957372685685,16.7380050975816,
1.23230418924702E-15));
#119155=CARTESIAN_POINT('Ctrl Pts',(-19.4773890628972,16.7675693190178,
-4.67334893926385E-15));
#119156=CARTESIAN_POINT('Ctrl Pts',(-19.5571491449815,16.8015339789002,
-1.47154927005622E-14));
#119157=CARTESIAN_POINT('Ctrl Pts',(-19.6348154881073,16.8395812463466,
-1.46480050311482E-14));
#119158=CARTESIAN_POINT('Ctrl Pts',(-19.7143271339384,16.8785324925657,
-1.45789138978149E-14));
#119159=CARTESIAN_POINT('Ctrl Pts',(-19.791645087401,16.921763301817,-1.99347487809546E-15));
#119160=CARTESIAN_POINT('Ctrl Pts',(-19.8665231354225,16.9689790854406,
-1.5404344466674E-15));
#119161=CARTESIAN_POINT('Ctrl Pts',(-19.9365885602911,17.0131601775965,
-1.1165122004366E-15));
#119162=CARTESIAN_POINT('Ctrl Pts',(-20.0045177778059,17.0608314259461,
-4.38762558481736E-15));
#119163=CARTESIAN_POINT('Ctrl Pts',(-20.0700782293505,17.1117789745462,
-6.47398801234544E-15));
#119164=CARTESIAN_POINT('Ctrl Pts',(-20.0997466327889,17.1348345269478,
-7.67905425978548E-15));
#119165=CARTESIAN_POINT('Ctrl Pts',(-20.1289294943527,17.1585613303937,
-2.17441215594909E-14));
#119166=CARTESIAN_POINT('Ctrl Pts',(-20.1576028725501,17.1829408480985,
-1.05609965217468E-14));
#119167=CARTESIAN_POINT('Ctrl Pts',(-20.1753080913464,17.197994696729,-3.771524073573E-15));
#119168=CARTESIAN_POINT('Ctrl Pts',(-20.192819023282,17.213297426603,2.39813803353757E-14));
#119169=CARTESIAN_POINT('Ctrl Pts',(-20.2101297182957,17.228844786453,1.88737914186277E-14));
#119170=CARTESIAN_POINT('Ctrl Pts',(-20.2222917522923,17.2397679480536,
1.53214174626332E-14));
#119171=CARTESIAN_POINT('Ctrl Pts',(-20.2343567224894,17.2508136607941,
1.04616494884397E-14));
#119172=CARTESIAN_POINT('Ctrl Pts',(-20.2463056670645,17.2619643610397,
1.13103970633688E-14));
#119173=CARTESIAN_POINT('Ctrl Pts',(-20.309737445094,17.3211586052181,1.46542491453268E-14));
#119174=CARTESIAN_POINT('Ctrl Pts',(-20.3700068842138,17.3834001964164,
1.3331333505949E-14));
#119175=CARTESIAN_POINT('Ctrl Pts',(-20.4268834249918,17.4484109388489,
4.71844785465692E-16));
#119176=CARTESIAN_POINT('Ctrl Pts',(-20.4830375676453,17.5125959693487,
-1.22243134931973E-14));
#119177=CARTESIAN_POINT('Ctrl Pts',(-20.5358849034902,17.5794810921953,
4.32698449193755E-15));
#119178=CARTESIAN_POINT('Ctrl Pts',(-20.5851610289878,17.6488247163806,
4.9960036108132E-15));
#119179=CARTESIAN_POINT('Ctrl Pts',(-20.6305982574028,17.712766068494,5.61290224501695E-15));
#119180=CARTESIAN_POINT('Ctrl Pts',(-20.6729989034471,17.7787984983198,
1.74504747378125E-14));
#119181=CARTESIAN_POINT('Ctrl Pts',(-20.7121179763249,17.8467438133767,
-5.41233724504764E-16));
#119182=CARTESIAN_POINT('Ctrl Pts',(-20.7284900279032,17.8751801775537,
-7.96914155170017E-15));
#119183=CARTESIAN_POINT('Ctrl Pts',(-20.7442868194365,17.9039516828061,
1.02457455428025E-15));
#119184=CARTESIAN_POINT('Ctrl Pts',(-20.7594882783128,17.9330455001009,
1.22540866343002E-14));
#119185=CARTESIAN_POINT('Ctrl Pts',(-20.7693449710067,17.9519100590029,
1.96618582104559E-14));
#119186=CARTESIAN_POINT('Ctrl Pts',(-20.7789513429732,17.970910128766,2.31589035439596E-14));
#119187=CARTESIAN_POINT('Ctrl Pts',(-20.7883016221878,17.9900422154472,
2.25791607633141E-14));
#119188=CARTESIAN_POINT('Ctrl Pts',(-20.7942275728048,18.0021676074567,
2.21995283693054E-14));
#119189=CARTESIAN_POINT('Ctrl Pts',(-20.8000468301417,18.0143382523374,
-7.82794172139843E-16));
#119190=CARTESIAN_POINT('Ctrl Pts',(-20.8057567255896,18.0265495880407,
-6.80011602582908E-16));
#119191=CARTESIAN_POINT('Ctrl Pts',(-20.8408822594586,18.1016699978184,
-4.24130062536125E-16));
#119192=CARTESIAN_POINT('Ctrl Pts',(-20.8718943559605,18.1783721483409,
-2.22042397420453E-14));
#119193=CARTESIAN_POINT('Ctrl Pts',(-20.8985462175416,18.2564274689474,
-7.57727214306669E-15));
#119194=CARTESIAN_POINT('Ctrl Pts',(-20.9251980791227,18.3344827895539,
7.49378466576201E-15));
#119195=CARTESIAN_POINT('Ctrl Pts',(-20.9474901778909,18.4138920100306,
4.88674281099961E-16));
#119196=CARTESIAN_POINT('Ctrl Pts',(-20.9651214076632,18.4944358221201,
-7.63278329429795E-15));
#119197=CARTESIAN_POINT('Ctrl Pts',(-20.9829513884047,18.5758875777237,
-1.55637816228118E-14));
#119198=CARTESIAN_POINT('Ctrl Pts',(-20.9960140913518,18.658500875996,1.15461163552663E-14));
#119199=CARTESIAN_POINT('Ctrl Pts',(-21.0043852377911,18.741883902842,4.69069227904129E-15));
#119200=CARTESIAN_POINT('Ctrl Pts',(-21.0073021823588,18.7709389037262,
2.30190453493397E-15));
#119201=CARTESIAN_POINT('Ctrl Pts',(-21.00964903562,18.8000872405097,2.61472081366534E-15));
#119202=CARTESIAN_POINT('Ctrl Pts',(-21.0114276099525,18.8293118127927,
5.68989300120393E-15));
#119203=CARTESIAN_POINT('Ctrl Pts',(-21.0124180861908,18.8455867830844,
7.40243597734682E-15));
#119204=CARTESIAN_POINT('Ctrl Pts',(-21.0132324466529,18.861889846349,1.06678997328114E-14));
#119205=CARTESIAN_POINT('Ctrl Pts',(-21.0138703004904,18.8781994766446,
7.41073868937292E-15));
#119206=CARTESIAN_POINT('Ctrl Pts',(-21.0156561554122,18.9238629685382,
-1.7086186600829E-15));
#119207=CARTESIAN_POINT('Ctrl Pts',(-21.0160589030104,18.9695495775744,
-5.36082417604155E-15));
#119208=CARTESIAN_POINT('Ctrl Pts',(-21.0151046780539,19.0152032729735,
-5.27355936696949E-16));
#119209=CARTESIAN_POINT('Ctrl Pts',(-21.0142961185276,19.0538877886947,
3.56826822819105E-15));
#119210=CARTESIAN_POINT('Ctrl Pts',(-21.0125130883006,19.0925470966385,
8.8757475914889E-15));
#119211=CARTESIAN_POINT('Ctrl Pts',(-21.0097683504117,19.1311426359222,
5.16253706450698E-15));
#119212=CARTESIAN_POINT('Ctrl Pts',(-21.0039587339496,19.2128354202505,
-2.62298544613293E-15));
#119213=CARTESIAN_POINT('Ctrl Pts',(-20.9938436162584,19.2942438410435,
-1.34729324233074E-14));
#119214=CARTESIAN_POINT('Ctrl Pts',(-20.9795069236666,19.3749917573276,
2.08166817117217E-15));
#119215=CARTESIAN_POINT('Ctrl Pts',(-20.9654095554313,19.4543917376786,
1.73766137054392E-14));
#119216=CARTESIAN_POINT('Ctrl Pts',(-20.9472298872587,19.5331539565538,
-1.43672378246897E-15));
#119217=CARTESIAN_POINT('Ctrl Pts',(-20.9250049246735,19.6108953906176,
-1.52655665885959E-15));
#119218=CARTESIAN_POINT('Ctrl Pts',(-20.9157258007275,19.6433531461548,
-1.56406270150217E-15));
#119219=CARTESIAN_POINT('Ctrl Pts',(-20.9057410485004,19.6756325821129,
-2.56785656981742E-15));
#119220=CARTESIAN_POINT('Ctrl Pts',(-20.8950514018658,19.7077039335531,
4.57966997657877E-15));
#119221=CARTESIAN_POINT('Ctrl Pts',(-20.8895107318069,19.72432719368,8.10553462204269E-15));
#119222=CARTESIAN_POINT('Ctrl Pts',(-20.8837798046829,19.7408965824585,
-8.47385102258745E-15));
#119223=CARTESIAN_POINT('Ctrl Pts',(-20.8778666060763,19.757386588617,-4.9960036108132E-15));
#119224=CARTESIAN_POINT('Ctrl Pts',(-20.8511334429462,19.8319367693201,
1.07200736924069E-14));
#119225=CARTESIAN_POINT('Ctrl Pts',(-20.8206474027028,19.9049627949995,
1.69200158934511E-14));
#119226=CARTESIAN_POINT('Ctrl Pts',(-20.7864673380873,19.9761054066943,
1.74860126378462E-14));
#119227=CARTESIAN_POINT('Ctrl Pts',(-20.7601551358713,20.0308717977514,
1.79217233645422E-14));
#119228=CARTESIAN_POINT('Ctrl Pts',(-20.7316529099465,20.0845216847886,
1.90313142705558E-16));
#119229=CARTESIAN_POINT('Ctrl Pts',(-20.7009723060731,20.1368764894501,
-6.60582699651968E-15));
#119230=CARTESIAN_POINT('Ctrl Pts',(-20.6917380360057,20.1526342759514,
-8.36889325698314E-15));
#119231=CARTESIAN_POINT('Ctrl Pts',(-20.6823063437492,20.1682746386422,
-7.8227685048287E-15));
#119232=CARTESIAN_POINT('Ctrl Pts',(-20.6726773354748,20.1837924272005,
6.38378239159465E-15));
#119233=CARTESIAN_POINT('Ctrl Pts',(-20.6644524181989,20.1970474295393,
1.8695920822413E-14));
#119234=CARTESIAN_POINT('Ctrl Pts',(-20.6560858012134,20.2102092325172,
-1.06494413537713E-14));
#119235=CARTESIAN_POINT('Ctrl Pts',(-20.64758209464,20.2232683236723,-1.08524300657109E-14));
#119236=CARTESIAN_POINT('Ctrl Pts',(-20.6064305700017,20.2864644731141,
-1.1070441092253E-14));
#119237=CARTESIAN_POINT('Ctrl Pts',(-20.5620419244788,20.3473056726972,
-5.11924385313933E-15));
#119238=CARTESIAN_POINT('Ctrl Pts',(-20.5144495335262,20.4054521925719,
-8.82627304576999E-15));
#119239=CARTESIAN_POINT('Ctrl Pts',(-20.4703173116583,20.4593712133354,
-1.25884914482375E-14));
#119240=CARTESIAN_POINT('Ctrl Pts',(-20.4234297145935,20.5109732585207,
9.12964091805133E-15));
#119241=CARTESIAN_POINT('Ctrl Pts',(-20.3737907847676,20.5599542646918,
6.32827124036339E-15));
#119242=CARTESIAN_POINT('Ctrl Pts',(-20.3682022242118,20.5654687534213,
6.19434691003275E-15));
#119243=CARTESIAN_POINT('Ctrl Pts',(-20.3625787693224,20.5709499818026,
2.24934943646516E-15));
#119244=CARTESIAN_POINT('Ctrl Pts',(-20.3569207886222,20.5763978007994,
-2.27595720048157E-15));
#119245=CARTESIAN_POINT('Ctrl Pts',(20.3504145334569,20.5721720813046,-0.0021418961558211));
#119246=CARTESIAN_POINT('Ctrl Pts',(20.8038322552136,20.0337689331937,-0.0445524877679966));
#119247=CARTESIAN_POINT('Ctrl Pts',(21.1220877011301,18.4777891502142,-0.12935501494065));
#119248=CARTESIAN_POINT('Ctrl Pts',(19.4066027174179,16.8027744939582,-0.256549477673783));
#119249=CARTESIAN_POINT('Ctrl Pts',(17.0746532806956,17.3436542441791,-0.383725284355217));
#119250=CARTESIAN_POINT('Ctrl Pts',(16.2649072910693,19.5945942026566,-0.510901091036651));
#119251=CARTESIAN_POINT('Ctrl Pts',(17.7204711796095,21.4952124979738,-0.638076897718085));
#119252=CARTESIAN_POINT('Ctrl Pts',(20.1058486786829,21.2993774626889,-0.765252704399521));
#119253=CARTESIAN_POINT('Ctrl Pts',(21.2326588902647,19.1880164416469,-0.892428511080953));
#119254=CARTESIAN_POINT('Ctrl Pts',(20.06709493847,17.0975178673283,-1.01960431776238));
#119255=CARTESIAN_POINT('Ctrl Pts',(17.6785041641668,16.9461239968056,-1.14678012444382));
#119256=CARTESIAN_POINT('Ctrl Pts',(16.2582626906796,18.8725530643131,-1.27395593112525));
#119257=CARTESIAN_POINT('Ctrl Pts',(17.1093578952725,21.1095174457448,-1.40113173780669));
#119258=CARTESIAN_POINT('Ctrl Pts',(19.4509606892502,21.6046936825495,-1.52830754448812));
#119259=CARTESIAN_POINT('Ctrl Pts',(21.1347969163821,19.9038129555627,-1.65548335116956));
#119260=CARTESIAN_POINT('Ctrl Pts',(20.6160507930577,17.5673149720866,-1.78265915785099));
#119261=CARTESIAN_POINT('Ctrl Pts',(18.3706399789337,16.7387982516159,-1.90983496453243));
#119262=CARTESIAN_POINT('Ctrl Pts',(16.4585893803026,18.1783720157104,-2.03701077121386));
#119263=CARTESIAN_POINT('Ctrl Pts',(16.6340868238919,20.5653184744001,-2.16418657789529));
#119264=CARTESIAN_POINT('Ctrl Pts',(18.7361242574646,21.709761474113,-2.29136238457673));
#119265=CARTESIAN_POINT('Ctrl Pts',(20.8362128238147,20.5617460765933,-2.41853819125816));
#119266=CARTESIAN_POINT('Ctrl Pts',(21.0076515986441,18.1745049051026,-2.54571399793959));
#119267=CARTESIAN_POINT('Ctrl Pts',(19.0931561523786,16.7381836953926,-2.67288980462103));
#119268=CARTESIAN_POINT('Ctrl Pts',(16.84915722705,17.5705179418497,-2.80006561130246));
#119269=CARTESIAN_POINT('Ctrl Pts',(16.3343845598861,19.9078926688087,-2.9272414179839));
#119270=CARTESIAN_POINT('Ctrl Pts',(18.021110121826,21.605911619971,-3.05441722466533));
#119271=CARTESIAN_POINT('Ctrl Pts',(20.3618679001945,21.1067478080081,-3.18159303134677));
#119272=CARTESIAN_POINT('Ctrl Pts',(21.2091579169385,18.8683530439058,-3.3087688380282));
#119273=CARTESIAN_POINT('Ctrl Pts',(19.7856441705552,16.9443155958186,-3.43594464470964));
#119274=CARTESIAN_POINT('Ctrl Pts',(17.3973121700664,17.0998204018171,-3.56312045139107));
#119275=CARTESIAN_POINT('Ctrl Pts',(16.2353082893486,19.1922014547983,-3.69029625807251));
#119276=CARTESIAN_POINT('Ctrl Pts',(17.3656989668499,21.3018290061115,-3.81747206475393));
#119277=CARTESIAN_POINT('Ctrl Pts',(19.7514209159292,21.4932507158639,-3.94464787143538));
#119278=CARTESIAN_POINT('Ctrl Pts',(21.2037223229058,19.5908490462334,-4.0718236781168));
#119279=CARTESIAN_POINT('Ctrl Pts',(20.390206786872,17.3399594527915,-4.19899948479825));
#119280=CARTESIAN_POINT('Ctrl Pts',(18.0572243196692,16.8056334315311,-4.32617529147967));
#119281=CARTESIAN_POINT('Ctrl Pts',(16.345141533734,18.4780819429591,-4.45335109816111));
#119282=CARTESIAN_POINT('Ctrl Pts',(16.8246881213196,20.8229372816948,-4.58052690484254));
#119283=CARTESIAN_POINT('Ctrl Pts',(19.0559098523345,21.6889402125877,-4.70770271152398));
#119284=CARTESIAN_POINT('Ctrl Pts',(20.9917992738112,20.2815867967456,-4.83487851820542));
#119285=CARTESIAN_POINT('Ctrl Pts',(20.8562979963933,17.8920364430003,-4.96205432488684));
#119286=CARTESIAN_POINT('Ctrl Pts',(18.7737200319539,16.7125532886911,-5.0892301315683));
#119287=CARTESIAN_POINT('Ctrl Pts',(16.6547014035,17.8252399209163,-5.21640593824971));
#119288=CARTESIAN_POINT('Ctrl Pts',(16.4433101815092,20.2092754157301,-5.34358174493116));
#119289=CARTESIAN_POINT('Ctrl Pts',(18.3334846917389,21.6774551765717,-5.47075755161258));
#119290=CARTESIAN_POINT('Ctrl Pts',(20.5911071385146,20.8828153983818,-5.59793335829403));
#119291=CARTESIAN_POINT('Ctrl Pts',(21.1449490507717,18.5543887567427,-5.72510916497545));
#119292=CARTESIAN_POINT('Ctrl Pts',(19.48689484932,16.8283621769022,-5.85228497165689));
#119293=CARTESIAN_POINT('Ctrl Pts',(17.1381063535418,17.2882579165725,-5.97946077833832));
#119294=CARTESIAN_POINT('Ctrl Pts',(16.2534512260582,19.5121501789549,-6.10663658501977));
#119295=CARTESIAN_POINT('Ctrl Pts',(17.6445456384458,21.4597558436343,-6.23381239170119));
#119296=CARTESIAN_POINT('Ctrl Pts',(20.0351468083957,21.3442675953078,-6.36098819838263));
#119297=CARTESIAN_POINT('Ctrl Pts',(21.2320265399213,19.271638733806,-6.48816400506407));
#119298=CARTESIAN_POINT('Ctrl Pts',(20.1371219660819,17.1433775977014,-6.6153398117455));
#119299=CARTESIAN_POINT('Ctrl Pts',(17.7549400759333,16.9120316845865,-6.74251561842693));
#119300=CARTESIAN_POINT('Ctrl Pts',(16.2709848988036,18.7898465107973,-6.86969142510836));
#119301=CARTESIAN_POINT('Ctrl Pts',(17.0466932050637,21.0540435236181,-6.99686723178981));
#119302=CARTESIAN_POINT('Ctrl Pts',(19.3704007696072,21.6273624957014,-7.12404303847125));
#119303=CARTESIAN_POINT('Ctrl Pts',(21.1102501275226,19.9838188543493,-7.25121884515265));
#119304=CARTESIAN_POINT('Ctrl Pts',(20.6700374801522,17.6312618806795,-7.37839465183411));
#119305=CARTESIAN_POINT('Ctrl Pts',(18.4536306087803,16.7280165818806,-7.50557045851553));
#119306=CARTESIAN_POINT('Ctrl Pts',(16.4944452521654,18.1027544578749,-7.63274626519699));
#119307=CARTESIAN_POINT('Ctrl Pts',(16.5899123742445,20.494238833293,-7.75992207187839));
#119308=CARTESIAN_POINT('Ctrl Pts',(18.6524468158679,21.7084312259493,-7.88709787855984));
#119309=CARTESIAN_POINT('Ctrl Pts',(20.7898012421711,20.6313854768606,-8.01427368524127));
#119310=CARTESIAN_POINT('Ctrl Pts',(21.0410856261975,18.2512242118175,-8.14144949192272));
#119311=CARTESIAN_POINT('Ctrl Pts',(19.175762142071,16.7515976620282,-8.26862529860413));
#119312=CARTESIAN_POINT('Ctrl Pts',(16.9051493114451,17.5083201096033,-8.39580110528559));
#119313=CARTESIAN_POINT('Ctrl Pts',(16.3123934762929,19.827145676385,-8.52297691196702));
#119314=CARTESIAN_POINT('Ctrl Pts',(17.9413113247901,21.580695827397,-8.65015271864845));
#119315=CARTESIAN_POINT('Ctrl Pts',(20.2974718329846,21.1601971366828,-8.77732852532987));
#119316=CARTESIAN_POINT('Ctrl Pts',(21.2192439744216,18.9514310538806,-8.90450433201132));
#119317=CARTESIAN_POINT('Ctrl Pts',(19.8609590209642,16.9808033684772,-9.03168013869275));
#119318=CARTESIAN_POINT('Ctrl Pts',(17.4687591127375,17.0562426708819,-9.1588559453742));
#119319=CARTESIAN_POINT('Ctrl Pts',(16.2373391888682,19.1085380834297,-9.28603175205561));
#119320=CARTESIAN_POINT('Ctrl Pts',(17.296450598966,21.2548359449271,-9.41320755873705));
#119321=CARTESIAN_POINT('Ctrl Pts',(19.6744243601341,21.526041181719,-9.54038336541849));
#119322=CARTESIAN_POINT('Ctrl Pts',(21.1896171401977,19.6733398219446,-9.66755917209992));
#119323=CARTESIAN_POINT('Ctrl Pts',(20.4519336069186,17.3964703715815,-9.79473497878134));
#119324=CARTESIAN_POINT('Ctrl Pts',(18.1381526162766,16.7843192328824,-9.9219107854628));
#119325=CARTESIAN_POINT('Ctrl Pts',(16.3710246177412,18.3984970812188,-10.0490865921442));
#119326=CARTESIAN_POINT('Ctrl Pts',(16.7717798696356,20.7580959279184,-10.1762623988257));
#119327=CARTESIAN_POINT('Ctrl Pts',(18.9727503020227,21.6983302843557,-10.3034382055071));
#119328=CARTESIAN_POINT('Ctrl Pts',(20.9546821508189,20.356593486025,-10.4306140121885));
#119329=CARTESIAN_POINT('Ctrl Pts',(20.8992759573175,17.9638457678171,-10.5577898188699));
#119330=CARTESIAN_POINT('Ctrl Pts',(18.8573634651597,16.7152846505155,-10.6849656255514));
#119331=CARTESIAN_POINT('Ctrl Pts',(16.7022726505182,17.7563874648017,-10.8121414322328));
#119332=CARTESIAN_POINT('Ctrl Pts',(16.411165575805,20.1320069966963,-10.9393172389142));
#119333=CARTESIAN_POINT('Ctrl Pts',(18.2511149139269,21.6626597732632,-11.0664930455957));
#119334=CARTESIAN_POINT('Ctrl Pts',(20.5340813472922,20.9440668750279,-11.1936688522771));
#119335=CARTESIAN_POINT('Ctrl Pts',(21.1655848701657,18.635492685216,-11.3208446589586));
#119336=CARTESIAN_POINT('Ctrl Pts',(19.5662601958398,16.854910736706,-11.44802046564));
#119337=CARTESIAN_POINT('Ctrl Pts',(17.2033884477244,17.2358944518762,-11.5751962723214));
#119338=CARTESIAN_POINT('Ctrl Pts',(16.2447577983548,19.4289149185742,-11.7023720790029));
#119339=CARTESIAN_POINT('Ctrl Pts',(17.5698523691992,21.4220119728056,-11.8295478856843));
#119340=CARTESIAN_POINT('Ctrl Pts',(19.9629801361526,21.3866427728676,-11.9567236923657));
#119341=CARTESIAN_POINT('Ctrl Pts',(21.2285949072958,19.3552563644432,-12.0838994990471));
#119342=CARTESIAN_POINT('Ctrl Pts',(20.2055736830169,17.191523695202,-12.2110753057286));
#119343=CARTESIAN_POINT('Ctrl Pts',(17.8324749407335,16.8805351927773,-12.33825111241));
#119344=CARTESIAN_POINT('Ctrl Pts',(16.2864694853713,18.7076035060207,-12.4654269190915));
#119345=CARTESIAN_POINT('Ctrl Pts',(16.9859213663049,20.9965068581799,-12.5926027257729));
#119346=CARTESIAN_POINT('Ctrl Pts',(19.2891268956574,21.647318489013,-12.7197785324543));
#119347=CARTESIAN_POINT('Ctrl Pts',(21.0830379533052,20.0629591211559,-12.8469543391357));
#119348=CARTESIAN_POINT('Ctrl Pts',(20.7218524865336,17.6969801381849,-12.9741301458172));
#119349=CARTESIAN_POINT('Ctrl Pts',(18.5369357434076,16.7200204077588,-13.1013059524986));
#119350=CARTESIAN_POINT('Ctrl Pts',(16.5328132245178,18.0283798455839,-13.2284817591801));
#119351=CARTESIAN_POINT('Ctrl Pts',(16.5481429510737,20.4217198734009,-13.3556575658615));
#119352=CARTESIAN_POINT('Ctrl Pts',(18.5688608504302,21.7042995631227,-13.4828333725429));
#119353=CARTESIAN_POINT('Ctrl Pts',(20.7410836698255,20.6994316553031,-13.6100091792244));
#119354=CARTESIAN_POINT('Ctrl Pts',(21.0719317958176,18.3290200862303,-13.7371849859058));
#119355=CARTESIAN_POINT('Ctrl Pts',(19.2578726075595,16.7677703461939,-13.8643607925872));
#119356=CARTESIAN_POINT('Ctrl Pts',(16.9631928170665,17.4480321695901,-13.9915365992687));
#119357=CARTESIAN_POINT('Ctrl Pts',(16.2931187082259,19.7457075552633,-14.1187124059501));
#119358=CARTESIAN_POINT('Ctrl Pts',(17.862401686409,21.5528219466762,-14.2458882126315));
#119359=CARTESIAN_POINT('Ctrl Pts',(20.2313220198197,21.211460051876,-14.373064019313));
#119360=CARTESIAN_POINT('Ctrl Pts',(21.2265423343311,19.0348002220335,-14.5002398259944));
#119361=CARTESIAN_POINT('Ctrl Pts',(19.9350097617186,17.0197927522835,-14.6274156326758));
#119362=CARTESIAN_POINT('Ctrl Pts',(17.5416252758018,17.0150819306535,-14.7545914393573));
#119363=CARTESIAN_POINT('Ctrl Pts',(16.2421705922151,19.0249896436024,-14.8817672460387));
#119364=CARTESIAN_POINT('Ctrl Pts',(17.2288147298954,21.2055503134414,-15.0089430527202));
#119365=CARTESIAN_POINT('Ctrl Pts',(19.5963729305628,21.5562348664518,-15.1361188594016));
#119366=CARTESIAN_POINT('Ctrl Pts',(21.1727574923393,19.7553119911849,-15.263294666083));
#119367=CARTESIAN_POINT('Ctrl Pts',(20.5117334212554,17.455016647818,-15.3904704727644));
#119368=CARTESIAN_POINT('Ctrl Pts',(18.2197492747497,16.7657270414598,-15.5176462794459));
#119369=CARTESIAN_POINT('Ctrl Pts',(16.3995582506614,18.3198236038057,-15.6448220861273));
#119370=CARTESIAN_POINT('Ctrl Pts',(16.7210726397956,20.6915191970147,-15.7719978928088));
#119371=CARTESIAN_POINT('Ctrl Pts',(18.8893229455551,21.7049303183475,-15.8991736994902));
#119372=CARTESIAN_POINT('Ctrl Pts',(20.915074089197,20.4303151633691,-16.0263495061716));
#119373=CARTESIAN_POINT('Ctrl Pts',(20.9398251287258,18.0370540252336,-16.153525312853));
#119374=CARTESIAN_POINT('Ctrl Pts',(18.9408685215966,16.7208154556417,-16.2807011195345));
#119375=CARTESIAN_POINT('Ctrl Pts',(16.7521228856109,17.6891666472147,-16.4078769262159));
#119376=CARTESIAN_POINT('Ctrl Pts',(16.3816264929107,20.0537054843378,-16.5350527328974));
#119377=CARTESIAN_POINT('Ctrl Pts',(18.1692867881987,21.6451143437821,-16.6622285395788));
#119378=CARTESIAN_POINT('Ctrl Pts',(20.4750364052595,21.003374370981,-16.7894043462602));
#119379=CARTESIAN_POINT('Ctrl Pts',(21.1834931814011,18.7172421601046,-16.9165801529417));
#119380=CARTESIAN_POINT('Ctrl Pts',(19.6446919963,16.8841021212645,-17.0437559596231));
#119381=CARTESIAN_POINT('Ctrl Pts',(17.2703874285137,17.1857464625939,-17.1709317663045));
#119382=CARTESIAN_POINT('Ctrl Pts',(16.2388565530248,19.3454352230824,-17.298107572986));
#119383=CARTESIAN_POINT('Ctrl Pts',(17.4964649240676,21.3817880103836,-17.4252833796674));
#119384=CARTESIAN_POINT('Ctrl Pts',(19.8894349171892,21.4265775324573,-17.5524591863489));
#119385=CARTESIAN_POINT('Ctrl Pts',(21.2223650881681,19.4387121827512,-17.6796349930303));
#119386=CARTESIAN_POINT('Ctrl Pts',(20.272374736109,17.2419350387839,-17.8068107997117));
#119387=CARTESIAN_POINT('Ctrl Pts',(17.9110210459731,16.8516527827758,-17.9339866063932));
#119388=CARTESIAN_POINT('Ctrl Pts',(16.3046994663247,18.6259251609712,-18.0611624130746));
#119389=CARTESIAN_POINT('Ctrl Pts',(16.9271103469226,20.9369673901283,-18.188338219756));
#119390=CARTESIAN_POINT('Ctrl Pts',(19.2072303360084,21.6645416644746,-18.3155140264374));
#119391=CARTESIAN_POINT('Ctrl Pts',(21.053190863776,20.1411437456081,-18.4426898331189));
#119392=CARTESIAN_POINT('Ctrl Pts',(20.7714377192819,17.764396671431,-18.5698656398003));
#119393=CARTESIAN_POINT('Ctrl Pts',(18.6204619249281,16.7148183647849,-18.6970414464817));
#119394=CARTESIAN_POINT('Ctrl Pts',(16.5736502676105,17.9553317781408,-18.8242172531632));
#119395=CARTESIAN_POINT('Ctrl Pts',(16.5088254030919,20.347842849113,-18.9513930598446));
#119396=CARTESIAN_POINT('Ctrl Pts',(18.4854601217909,21.6973711671814,-19.078568866526));
#119397=CARTESIAN_POINT('Ctrl Pts',(20.6901147517246,20.7658082595486,-19.2057446732075));
#119398=CARTESIAN_POINT('Ctrl Pts',(21.100155508854,18.4078052787827,-19.3329204798889));
#119399=CARTESIAN_POINT('Ctrl Pts',(19.3393954434521,16.786683597609,-19.4600962865703));
#119400=CARTESIAN_POINT('Ctrl Pts',(17.02322264018,17.3897217556752,-19.5872720932518));
#119401=CARTESIAN_POINT('Ctrl Pts',(16.2765818693588,19.6636696421892,-19.7144478999332));
#119402=CARTESIAN_POINT('Ctrl Pts',(17.7844697326546,21.5223212653023,-19.8416237066147));
#119403=CARTESIAN_POINT('Ctrl Pts',(20.1634926358433,21.2604790121031,-19.9687995132961));
#119404=CARTESIAN_POINT('Ctrl Pts',(21.231044858401,19.1183671093666,-20.0959753199775));
#119405=CARTESIAN_POINT('Ctrl Pts',(20.0077132370737,17.0612398664333,-20.2231511266589));
#119406=CARTESIAN_POINT('Ctrl Pts',(17.6158291045619,16.976384633048,-20.3503269333404));
#119407=CARTESIAN_POINT('Ctrl Pts',(16.2497967346393,18.9416493085074,-20.4775027400218));
#119408=CARTESIAN_POINT('Ctrl Pts',(17.1628678921721,21.1540284415978,-20.6046785467032));
#119409=CARTESIAN_POINT('Ctrl Pts',(19.5173528955041,21.5837958860619,-20.7318543533847));
#119410=CARTESIAN_POINT('Ctrl Pts',(21.1531647607153,19.8366774894172,-20.8590301600661));
#119411=CARTESIAN_POINT('Ctrl Pts',(20.5695343937816,17.5155251277943,-20.9862059667476));
#119412=CARTESIAN_POINT('Ctrl Pts',(18.301931936395,16.7498921279798,-21.113381773429));
#119413=CARTESIAN_POINT('Ctrl Pts',(16.430692762331,18.2421219844588,-21.2405575801104));
#119414=CARTESIAN_POINT('Ctrl Pts',(16.6726573424412,20.6233352795928,-21.3677333867919));
#119415=CARTESIAN_POINT('Ctrl Pts',(18.8056557941431,21.7086298106478,-21.4949091934733));
#119416=CARTESIAN_POINT('Ctrl Pts',(20.8731458549779,20.5028678015929,-21.6220850001547));
#119417=CARTESIAN_POINT('Ctrl Pts',(20.9776565334948,18.111196073242,-21.7492608068362));
#119418=CARTESIAN_POINT('Ctrl Pts',(19.0246114642159,16.7298799538284,-21.8764366135176));
#119419=CARTESIAN_POINT('Ctrl Pts',(16.8032831853607,17.6222026293144,-22.0036124201991));
#119420=CARTESIAN_POINT('Ctrl Pts',(16.3565572075883,19.9774759742341,-22.1307882268804));
#119421=CARTESIAN_POINT('Ctrl Pts',(17.5080922618947,21.070504731278,-22.2155720980014));
#119422=CARTESIAN_POINT('Ctrl Pts',(18.1877583250969,21.2523734297384,-22.2579640335619));
#119423=CARTESIAN_POINT('Ctrl Pts',(20.4651728790455,20.6688093317616,0.084476493734548));
#119424=CARTESIAN_POINT('Ctrl Pts',(20.9507812712845,20.0921819204693,0.0420659021223723));
#119425=CARTESIAN_POINT('Ctrl Pts',(21.2916314586439,18.4257343942419,-0.0427366250502812));
#119426=CARTESIAN_POINT('Ctrl Pts',(19.4543545616952,16.6318010405789,-0.169931087783413));
#119427=CARTESIAN_POINT('Ctrl Pts',(16.9568469381246,17.2110808818736,-0.297106894464847));
#119428=CARTESIAN_POINT('Ctrl Pts',(16.0896125331239,19.6218277093859,-0.424282701146282));
#119429=CARTESIAN_POINT('Ctrl Pts',(17.6485150766254,21.6573815714476,-0.551458507827716));
#119430=CARTESIAN_POINT('Ctrl Pts',(20.203243920748,21.4476431071891,-0.67863431450915));
#119431=CARTESIAN_POINT('Ctrl Pts',(21.410052717468,19.1863847097626,-0.805810121190585));
#119432=CARTESIAN_POINT('Ctrl Pts',(20.1617388348746,16.9474699013169,-0.932985927872018));
#119433=CARTESIAN_POINT('Ctrl Pts',(17.6035685870678,16.7853277296908,-1.06016173455346));
#119434=CARTESIAN_POINT('Ctrl Pts',(16.0824961952363,18.8485248156151,-1.18733754123489));
#119435=CARTESIAN_POINT('Ctrl Pts',(16.994015428193,21.2443038613797,-1.31451334791632));
#119436=CARTESIAN_POINT('Ctrl Pts',(19.5018617550643,21.7746354401676,-1.44168915459776));
#119437=CARTESIAN_POINT('Ctrl Pts',(21.3052429724622,19.9529996381475,-1.56886496127919));
#119438=CARTESIAN_POINT('Ctrl Pts',(20.7496681485408,17.4506205409442,-1.69604076796063));
#119439=CARTESIAN_POINT('Ctrl Pts',(18.3448430103915,16.5632827654992,-1.82321657464206));
#119440=CARTESIAN_POINT('Ctrl Pts',(16.2970452015994,18.1050599558195,-1.9503923813235));
#119441=CARTESIAN_POINT('Ctrl Pts',(16.4850021943108,20.6614691488127,-2.07756818800493));
#119442=CARTESIAN_POINT('Ctrl Pts',(18.736275070432,21.8871625843198,-2.20474399468636));
#119443=CARTESIAN_POINT('Ctrl Pts',(20.9854607183013,20.6576431264228,-2.3319198013678));
#119444=CARTESIAN_POINT('Ctrl Pts',(21.1690708945641,18.1009182973116,-2.45909560804923));
#119445=CARTESIAN_POINT('Ctrl Pts',(19.1186546646734,16.5626245784783,-2.58627141473067));
#119446=CARTESIAN_POINT('Ctrl Pts',(16.7153416532344,17.4540509075189,-2.7134472214121));
#119447=CARTESIAN_POINT('Ctrl Pts',(16.1640223834416,19.9573689931488,-2.84062302809354));
#119448=CARTESIAN_POINT('Ctrl Pts',(17.9704980657522,21.7759398458068,-2.96779883477497));
#119449=CARTESIAN_POINT('Ctrl Pts',(20.4774393846103,21.2413375915055,-3.0949746414564));
#119450=CARTESIAN_POINT('Ctrl Pts',(21.3848832780629,18.8440266121716,-3.22215044813784));
#119451=CARTESIAN_POINT('Ctrl Pts',(19.8603062963049,16.7833909401617,-3.34932625481927));
#119452=CARTESIAN_POINT('Ctrl Pts',(17.3024131941191,16.9499359056603,-3.4765020615007));
#119453=CARTESIAN_POINT('Ctrl Pts',(16.0579121320417,19.1908668405009,-3.60367786818214));
#119454=CARTESIAN_POINT('Ctrl Pts',(17.268555592065,21.4502686994473,-3.73085367486357));
#119455=CARTESIAN_POINT('Ctrl Pts',(19.8236533406339,21.6552805114082,-3.85802948154501));
#119456=CARTESIAN_POINT('Ctrl Pts',(21.3790617806833,19.6178166632753,-3.98520528822644));
#119457=CARTESIAN_POINT('Ctrl Pts',(20.5077902080058,17.2071237764952,-4.11238109490788));
#119458=CARTESIAN_POINT('Ctrl Pts',(18.0091762133191,16.634862950186,-4.23955690158931));
#119459=CARTESIAN_POINT('Ctrl Pts',(16.1755430552745,18.4260479739882,-4.36673270827075));
#119460=CARTESIAN_POINT('Ctrl Pts',(16.6891353482686,20.9373777620364,-4.49390851495218));
#119461=CARTESIAN_POINT('Ctrl Pts',(19.0787640406122,21.8648631045058,-4.62108432163361));
#119462=CARTESIAN_POINT('Ctrl Pts',(21.1520931241638,20.3575937659115,-4.74826012831505));
#119463=CARTESIAN_POINT('Ctrl Pts',(21.0069718500806,17.7983958127287,-4.87543593499648));
#119464=CARTESIAN_POINT('Ctrl Pts',(18.7765399800919,16.5351745252634,-5.00261174167792));
#119465=CARTESIAN_POINT('Ctrl Pts',(16.5070803186978,17.7268570304097,-5.12978754835935));
#119466=CARTESIAN_POINT('Ctrl Pts',(16.280681246675,20.2801485938535,-5.25696335504078));
#119467=CARTESIAN_POINT('Ctrl Pts',(18.305049860693,21.8525626812824,-5.38413916172222));
#119468=CARTESIAN_POINT('Ctrl Pts',(20.722953603877,21.0015069625052,-5.51131496840365));
#119469=CARTESIAN_POINT('Ctrl Pts',(21.3161158638869,18.5077722370249,-5.63849077508509));
#119470=CARTESIAN_POINT('Ctrl Pts',(19.5403470829654,16.6592053368368,-5.76566658176652));
#119471=CARTESIAN_POINT('Ctrl Pts',(17.0248049009675,17.1517516578618,-5.89284238844796));
#119472=CARTESIAN_POINT('Ctrl Pts',(16.0773431377199,19.5335305214322,-6.02001819512939));
#119473=CARTESIAN_POINT('Ctrl Pts',(17.5671991548932,21.6194076500902,-6.14719400181082));
#119474=CARTESIAN_POINT('Ctrl Pts',(20.127522527624,21.4957202424278,-6.27436980849226));
#119475=CARTESIAN_POINT('Ctrl Pts',(21.4093754730223,19.2759438180688,-6.40154561517369));
#119476=CARTESIAN_POINT('Ctrl Pts',(20.2367374744517,16.9965854714996,-6.52872142185513));
#119477=CARTESIAN_POINT('Ctrl Pts',(17.6854311134782,16.7488150127633,-6.65589722853656));
#119478=CARTESIAN_POINT('Ctrl Pts',(16.0961216243634,18.7599464593815,-6.78307303521799));
#119479=CARTESIAN_POINT('Ctrl Pts',(16.9269018196985,21.1848915339771,-6.91024884189944));
#119480=CARTESIAN_POINT('Ctrl Pts',(19.4155824342976,21.7989136396743,-7.03742464858086));
#119481=CARTESIAN_POINT('Ctrl Pts',(21.2789534692056,20.0386856050059,-7.1646004552623));
#119482=CARTESIAN_POINT('Ctrl Pts',(20.8074876537439,17.5191073997068,-7.29177626194374));
#119483=CARTESIAN_POINT('Ctrl Pts',(18.4337256111302,16.551735644479,-7.41895206862516));
#119484=CARTESIAN_POINT('Ctrl Pts',(16.335446683174,18.0240738828814,-7.54612787530661));
#119485=CARTESIAN_POINT('Ctrl Pts',(16.4376915523973,20.5853431647969,-7.67330368198803));
#119486=CARTESIAN_POINT('Ctrl Pts',(18.64665689732,21.8857378943683,-7.80047948866947));
#119487=CARTESIAN_POINT('Ctrl Pts',(20.9357541178272,20.7322266188132,-7.92765529535091));
#119488=CARTESIAN_POINT('Ctrl Pts',(21.2048785915005,18.1830843384694,-8.05483110203234));
#119489=CARTESIAN_POINT('Ctrl Pts',(19.2071253174932,16.5769908779387,-8.18200690871378));
#119490=CARTESIAN_POINT('Ctrl Pts',(16.7753089301549,17.3874373018554,-8.3091827153952));
#119491=CARTESIAN_POINT('Ctrl Pts',(16.1404700293211,19.8708893182541,-8.43635852207665));
#119492=CARTESIAN_POINT('Ctrl Pts',(17.8850339039608,21.7489338425049,-8.56353432875807));
#119493=CARTESIAN_POINT('Ctrl Pts',(20.4084714789379,21.2985815881968,-8.69071013543951));
#119494=CARTESIAN_POINT('Ctrl Pts',(21.3956854014105,18.9330027966444,-8.81788594212095));
#119495=CARTESIAN_POINT('Ctrl Pts',(19.9409681709163,16.8224691847183,-8.94506174880238));
#119496=CARTESIAN_POINT('Ctrl Pts',(17.3789325564997,16.9032643468714,-9.07223755548381));
#119497=CARTESIAN_POINT('Ctrl Pts',(16.0600872165237,19.1012637365415,-9.19941336216525));
#119498=CARTESIAN_POINT('Ctrl Pts',(17.1943908936429,21.3999393369342,-9.32658916884668));
#119499=CARTESIAN_POINT('Ctrl Pts',(19.7411903669265,21.6903989565872,-9.45376497552812));
#119500=CARTESIAN_POINT('Ctrl Pts',(21.3639551918393,19.7061639224262,-9.58094078220955));
#119501=CARTESIAN_POINT('Ctrl Pts',(20.5738993616681,17.2676467227782,-9.70811658889098));
#119502=CARTESIAN_POINT('Ctrl Pts',(18.0958500641997,16.6120355368737,-9.83529239557241));
#119503=CARTESIAN_POINT('Ctrl Pts',(16.2032637247762,18.3408129359606,-9.96246820225386));
#119504=CARTESIAN_POINT('Ctrl Pts',(16.6324708426624,20.8679329564033,-10.0896440089353));
#119505=CARTESIAN_POINT('Ctrl Pts',(18.989700526796,21.8749198302035,-10.2168198156167));
#119506=CARTESIAN_POINT('Ctrl Pts',(21.1123408481587,20.4379256013037,-10.3439956222982));
#119507=CARTESIAN_POINT('Ctrl Pts',(21.0530010578169,17.8753032847989,-10.4711714289796));
#119508=CARTESIAN_POINT('Ctrl Pts',(18.8661217303663,16.5380998018032,-10.5983472356611));
#119509=CARTESIAN_POINT('Ctrl Pts',(16.5580289157041,17.6531163517569,-10.7255230423425));
#119510=CARTESIAN_POINT('Ctrl Pts',(16.2462545148863,20.1973944558094,-10.8526988490239));
#119511=CARTESIAN_POINT('Ctrl Pts',(18.2168321897617,21.8367168692014,-10.9798746557054));
#119512=CARTESIAN_POINT('Ctrl Pts',(20.6618792314763,21.0671070254696,-11.1070504623868));
#119513=CARTESIAN_POINT('Ctrl Pts',(21.3382167359914,18.5946341888639,-11.2342262690682));
#119514=CARTESIAN_POINT('Ctrl Pts',(19.6253470211541,16.6876387279989,-11.3614020757497));
#119515=CARTESIAN_POINT('Ctrl Pts',(17.0947217376433,17.0956706167312,-11.4885778824311));
#119516=CARTESIAN_POINT('Ctrl Pts',(16.0680325147611,19.4443859224641,-11.6157536891125));
#119517=CARTESIAN_POINT('Ctrl Pts',(17.487202990982,21.5789841299002,-11.742929495794));
#119518=CARTESIAN_POINT('Ctrl Pts',(20.0502323380272,21.5411038718235,-11.8701053024754));
#119519=CARTESIAN_POINT('Ctrl Pts',(21.4057002095246,19.3654979339054,-11.9972811091568));
#119520=CARTESIAN_POINT('Ctrl Pts',(20.3100489631999,17.0481497308524,-12.1244569158383));
#119521=CARTESIAN_POINT('Ctrl Pts',(17.7684706137698,16.715082408115,-12.2516327225197));
#119522=CARTESIAN_POINT('Ctrl Pts',(16.1127055486938,18.6718645618152,-12.3788085292011));
#119523=CARTESIAN_POINT('Ctrl Pts',(16.8618154468087,21.1232700175309,-12.5059843358826));
#119524=CARTESIAN_POINT('Ctrl Pts',(19.3285384715983,21.8202864210249,-12.633160142564));
#119525=CARTESIAN_POINT('Ctrl Pts',(21.2498093499156,20.1234444838084,-12.7603359492454));
#119526=CARTESIAN_POINT('Ctrl Pts',(20.8629812984238,17.5894913653894,-12.8875117559269));
#119527=CARTESIAN_POINT('Ctrl Pts',(18.5229450451101,16.5431717770494,-13.0146875626083));
#119528=CARTESIAN_POINT('Ctrl Pts',(16.37653861336,17.9444189991727,-13.1418633692897));
#119529=CARTESIAN_POINT('Ctrl Pts',(16.3929566832965,20.5076756766722,-13.2690391759712));
#119530=CARTESIAN_POINT('Ctrl Pts',(18.5571366947732,21.8813129015941,-13.3962149826526));
#119531=CARTESIAN_POINT('Ctrl Pts',(20.8835778114207,20.8051037776138,-13.523390789334));
#119532=CARTESIAN_POINT('Ctrl Pts',(21.2379147039354,18.2664033789119,-13.6505665960155));
#119533=CARTESIAN_POINT('Ctrl Pts',(19.2950652660628,16.5943117517799,-13.7777424026969));
#119534=CARTESIAN_POINT('Ctrl Pts',(16.8374732702154,17.3228691824008,-13.9049182093783));
#119535=CARTESIAN_POINT('Ctrl Pts',(16.119826837221,19.7836694475537,-14.0320940160598));
#119536=CARTESIAN_POINT('Ctrl Pts',(17.800522027191,21.7190810384507,-14.1592698227412));
#119537=CARTESIAN_POINT('Ctrl Pts',(20.337625319036,21.3534839456345,-14.2864456294226));
#119538=CARTESIAN_POINT('Ctrl Pts',(21.4035019128779,19.0222908102495,-14.4136214361041));
#119539=CARTESIAN_POINT('Ctrl Pts',(20.0202761896291,16.8642266438473,-14.5407972427855));
#119540=CARTESIAN_POINT('Ctrl Pts',(17.4569718976996,16.8591813745337,-14.667973049467));
#119541=CARTESIAN_POINT('Ctrl Pts',(16.0652616283277,19.011783723759,-14.7951488561484));
#119542=CARTESIAN_POINT('Ctrl Pts',(17.1219531743809,21.347154641679,-14.9223246628298));
#119543=CARTESIAN_POINT('Ctrl Pts',(19.6575976280295,21.7227362605683,-15.0495004695112));
#119544=CARTESIAN_POINT('Ctrl Pts',(21.3458985828949,19.7939557563202,-15.1766762761927));
#119545=CARTESIAN_POINT('Ctrl Pts',(20.6379447006631,17.3303495279633,-15.3038520828741));
#119546=CARTESIAN_POINT('Ctrl Pts',(18.1832397277084,16.5921233813674,-15.4310278895556));
#119547=CARTESIAN_POINT('Ctrl Pts',(16.2338231205434,18.2565539865522,-15.558203696237));
#119548=CARTESIAN_POINT('Ctrl Pts',(16.5781636218018,20.7966295694748,-15.6853795029184));
#119549=CARTESIAN_POINT('Ctrl Pts',(18.9003501937609,21.8819884376745,-15.8125553095998));
#119550=CARTESIAN_POINT('Ctrl Pts',(21.0699207878016,20.5168811945468,-15.9397311162813));
#119551=CARTESIAN_POINT('Ctrl Pts',(21.0964290426296,17.9537090075503,-16.0669069229627));
#119552=CARTESIAN_POINT('Ctrl Pts',(18.9555552797279,16.5440232698465,-16.1940827296442));
#119553=CARTESIAN_POINT('Ctrl Pts',(16.6114182989473,17.5811231508143,-16.3212585363256));
#119554=CARTESIAN_POINT('Ctrl Pts',(16.2146182866043,20.1135338793437,-16.448434343007));
#119555=CARTESIAN_POINT('Ctrl Pts',(18.1291946258374,21.8179257911455,-16.5756101496885));
#119556=CARTESIAN_POINT('Ctrl Pts',(20.5986423574096,21.1306250936339,-16.7027859563699));
#119557=CARTESIAN_POINT('Ctrl Pts',(21.3573964588152,18.6821875180837,-16.8299617630513));
#119558=CARTESIAN_POINT('Ctrl Pts',(19.7093471356056,16.7189025728874,-16.9571375697328));
#119559=CARTESIAN_POINT('Ctrl Pts',(17.1664773523482,17.0419623400562,-17.0843133764142));
#119560=CARTESIAN_POINT('Ctrl Pts',(16.0617123068835,19.3549795345634,-17.2114891830956));
#119561=CARTESIAN_POINT('Ctrl Pts',(17.4086053589731,21.5359044424863,-17.3386649897771));
#119562=CARTESIAN_POINT('Ctrl Pts',(19.9714657309362,21.5838738242719,-17.4658407964585));
#119563=CARTESIAN_POINT('Ctrl Pts',(21.3990281005501,19.4548787494468,-17.5930166031399));
#119564=CARTESIAN_POINT('Ctrl Pts',(20.3815925982089,17.1021400588277,-17.7201924098214));
#119565=CARTESIAN_POINT('Ctrl Pts',(17.8525931481391,16.6841494736224,-17.8473682165028));
#119566=CARTESIAN_POINT('Ctrl Pts',(16.1322297783753,18.5843874123414,-17.9745440231842));
#119567=CARTESIAN_POINT('Ctrl Pts',(16.7988291028752,21.0595035082658,-18.1017198298657));
#119568=CARTESIAN_POINT('Ctrl Pts',(19.240827615245,21.8387323664388,-18.2288956365471));
#119569=CARTESIAN_POINT('Ctrl Pts',(21.2178432478782,20.2071798738389,-18.3560714432285));
#119570=CARTESIAN_POINT('Ctrl Pts',(20.9160868653179,17.661694176945,-18.48324724991));
#119571=CARTESIAN_POINT('Ctrl Pts',(18.6124012193438,16.53760041183,-18.6104230565914));
#119572=CARTESIAN_POINT('Ctrl Pts',(16.4202749074846,17.8661848391805,-18.7375988632728));
#119573=CARTESIAN_POINT('Ctrl Pts',(16.3508477617745,20.4285537075334,-18.8647746699543));
#119574=CARTESIAN_POINT('Ctrl Pts',(18.4678148800254,21.8738926199146,-18.9919504766357));
#119575=CARTESIAN_POINT('Ctrl Pts',(20.8289903235801,20.8761928297688,-19.1191262833172));
#119576=CARTESIAN_POINT('Ctrl Pts',(21.2681421768659,18.3507819747449,-19.2463020899985));
#119577=CARTESIAN_POINT('Ctrl Pts',(19.3823758659115,16.6145677611307,-19.37347789668));
#119578=CARTESIAN_POINT('Ctrl Pts',(16.901764947602,17.260418984728,-19.5006537033614));
#119579=CARTESIAN_POINT('Ctrl Pts',(16.1021159552911,19.6958072023018,-19.6278295100429));
#119580=CARTESIAN_POINT('Ctrl Pts',(17.71705724637,21.6864149424128,-19.7550053167243));
#119581=CARTESIAN_POINT('Ctrl Pts',(20.2649803461583,21.4059830371408,-19.8821811234057));
#119582=CARTESIAN_POINT('Ctrl Pts',(21.4083240964178,19.11179058023,-20.0093569300872));
#119583=CARTESIAN_POINT('Ctrl Pts',(20.0981412930058,16.9086163213996,-20.1365327367686));
#119584=CARTESIAN_POINT('Ctrl Pts',(17.5364438729955,16.8177367384453,-20.2637085434501));
#119585=CARTESIAN_POINT('Ctrl Pts',(16.0734291934315,18.9225265902324,-20.3908843501315));
#119586=CARTESIAN_POINT('Ctrl Pts',(17.051324400287,21.2919749428039,-20.5180601568129));
#119587=CARTESIAN_POINT('Ctrl Pts',(19.5729675169019,21.7522539917445,-20.6452359634943));
#119588=CARTESIAN_POINT('Ctrl Pts',(21.3249148532192,19.8810978482246,-20.7724117701758));
#119589=CARTESIAN_POINT('Ctrl Pts',(20.6998492888418,17.3951538447513,-20.8995875768572));
#119590=CARTESIAN_POINT('Ctrl Pts',(18.2712569980454,16.5751642584499,-21.0267633835387));
#119591=CARTESIAN_POINT('Ctrl Pts',(16.2671680460494,18.173335892872,-21.1539391902201));
#119592=CARTESIAN_POINT('Ctrl Pts',(16.5263110505858,20.7236048928311,-21.2811149969015));
#119593=CARTESIAN_POINT('Ctrl Pts',(18.8107430413917,21.8859505777098,-21.408290803583));
#119594=CARTESIAN_POINT('Ctrl Pts',(21.0250158327644,20.594584752017,-21.5354666102644));
#119595=CARTESIAN_POINT('Ctrl Pts',(21.1369463112861,18.033114815932,-21.6626424169459));
#119596=CARTESIAN_POINT('Ctrl Pts',(19.045243604148,16.5537313076661,-21.7898182236272));
#119597=CARTESIAN_POINT('Ctrl Pts',(16.6662107556949,17.5094049812102,-21.9169940303087));
#119598=CARTESIAN_POINT('Ctrl Pts',(16.1877691919268,20.0318924082093,-22.0441698369901));
#119599=CARTESIAN_POINT('Ctrl Pts',(17.4210581868123,21.2025214152156,-22.1289537081111));
#119600=CARTESIAN_POINT('Ctrl Pts',(18.1489775608771,21.3973019939627,-22.1713456436716));
#119601=CARTESIAN_POINT('Ctrl Pts',(20.579931224634,20.7654465822185,0.171094883624917));
#119602=CARTESIAN_POINT('Ctrl Pts',(21.0977302873553,20.150594907745,0.128684292012742));
#119603=CARTESIAN_POINT('Ctrl Pts',(21.4611752161576,18.3736796382696,0.0438817648400879));
#119604=CARTESIAN_POINT('Ctrl Pts',(19.5021064059726,16.4608275871995,-0.0833126978930439));
#119605=CARTESIAN_POINT('Ctrl Pts',(16.8390405955535,17.0785075195682,-0.210488504574479));
#119606=CARTESIAN_POINT('Ctrl Pts',(15.9143177751785,19.6490612161152,-0.337664311255912));
#119607=CARTESIAN_POINT('Ctrl Pts',(17.5765589736414,21.8195506449214,-0.464840117937347));
#119608=CARTESIAN_POINT('Ctrl Pts',(20.300639162813,21.5959087516894,-0.592015924618781));
#119609=CARTESIAN_POINT('Ctrl Pts',(21.5874465446713,19.1847529778785,-0.719191731300216));
#119610=CARTESIAN_POINT('Ctrl Pts',(20.2563827312793,16.7974219353056,-0.84636753798165));
#119611=CARTESIAN_POINT('Ctrl Pts',(17.5286330099687,16.6245314625761,-0.973543344663085));
#119612=CARTESIAN_POINT('Ctrl Pts',(15.9067296997928,18.8244965669171,-1.10071915134451));
#119613=CARTESIAN_POINT('Ctrl Pts',(16.8786729611136,21.3790902770145,-1.22789495802595));
#119614=CARTESIAN_POINT('Ctrl Pts',(19.5527628208785,21.9445771977858,-1.35507076470738));
#119615=CARTESIAN_POINT('Ctrl Pts',(21.4756890285423,20.0021863207324,-1.48224657138883));
#119616=CARTESIAN_POINT('Ctrl Pts',(20.8832855040238,17.3339261098018,-1.60942237807025));
#119617=CARTESIAN_POINT('Ctrl Pts',(18.3190460418495,16.3877672793826,-1.73659818475169));
#119618=CARTESIAN_POINT('Ctrl Pts',(16.1355010228962,18.0317478959284,-1.86377399143312));
#119619=CARTESIAN_POINT('Ctrl Pts',(16.3359175647298,20.7576198232253,-1.99094979811455));
#119620=CARTESIAN_POINT('Ctrl Pts',(18.7364258833992,22.0645636945266,-2.11812560479599));
#119621=CARTESIAN_POINT('Ctrl Pts',(21.1347086127881,20.7535401762524,-2.24530141147742));
#119622=CARTESIAN_POINT('Ctrl Pts',(21.3304901904839,18.0273316895207,-2.37247721815887));
#119623=CARTESIAN_POINT('Ctrl Pts',(19.1441531769682,16.387065461564,-2.49965302484029));
#119624=CARTESIAN_POINT('Ctrl Pts',(16.5815260794188,17.337583873188,-2.62682883152173));
#119625=CARTESIAN_POINT('Ctrl Pts',(15.9936602069971,20.0068453174889,-2.75400463820316));
#119626=CARTESIAN_POINT('Ctrl Pts',(17.9198860096782,21.9459680716425,-2.88118044488459));
#119627=CARTESIAN_POINT('Ctrl Pts',(20.5930108690263,21.3759273750031,-3.00835625156604));
#119628=CARTESIAN_POINT('Ctrl Pts',(21.5606086391872,18.8197001804373,-3.13553205824747));
#119629=CARTESIAN_POINT('Ctrl Pts',(19.9349684220548,16.6224662845049,-3.2627078649289));
#119630=CARTESIAN_POINT('Ctrl Pts',(17.2075142181716,16.8000514095034,-3.38988367161033));
#119631=CARTESIAN_POINT('Ctrl Pts',(15.8805159747347,19.1895322262035,-3.51705947829178));
#119632=CARTESIAN_POINT('Ctrl Pts',(17.1714122172801,21.5987083927831,-3.6442352849732));
#119633=CARTESIAN_POINT('Ctrl Pts',(19.8958857653384,21.8173103069526,-3.77141109165464));
#119634=CARTESIAN_POINT('Ctrl Pts',(21.5544012384607,19.6447842803171,-3.89858689833607));
#119635=CARTESIAN_POINT('Ctrl Pts',(20.6253736291394,17.074288100199,-4.02576270501751));
#119636=CARTESIAN_POINT('Ctrl Pts',(17.961128106969,16.464092468841,-4.15293851169893));
#119637=CARTESIAN_POINT('Ctrl Pts',(16.0059445768151,18.3740140050173,-4.28011431838038));
#119638=CARTESIAN_POINT('Ctrl Pts',(16.5535825752176,21.0518182423779,-4.4072901250618));
#119639=CARTESIAN_POINT('Ctrl Pts',(19.10161822889,22.0407859964237,-4.53446593174325));
#119640=CARTESIAN_POINT('Ctrl Pts',(21.3123869745163,20.4336007350771,-4.66164173842467));
#119641=CARTESIAN_POINT('Ctrl Pts',(21.1576457037679,17.7047551824572,-4.78881754510611));
#119642=CARTESIAN_POINT('Ctrl Pts',(18.7793599282299,16.3577957618358,-4.91599335178755));
#119643=CARTESIAN_POINT('Ctrl Pts',(16.3594592338956,17.6284741399031,-5.04316915846898));
#119644=CARTESIAN_POINT('Ctrl Pts',(16.1180523118408,20.3510217719769,-5.17034496515041));
#119645=CARTESIAN_POINT('Ctrl Pts',(18.2766150296472,22.0276701859931,-5.29752077183185));
#119646=CARTESIAN_POINT('Ctrl Pts',(20.8548000692393,21.1201985266286,-5.42469657851328));
#119647=CARTESIAN_POINT('Ctrl Pts',(21.4872826770021,18.4611557173071,-5.55187238519472));
#119648=CARTESIAN_POINT('Ctrl Pts',(19.5937993166108,16.4900484967713,-5.67904819187615));
#119649=CARTESIAN_POINT('Ctrl Pts',(16.9115034483931,17.0152453991512,-5.80622399855758));
#119650=CARTESIAN_POINT('Ctrl Pts',(15.9012350493816,19.5549108639094,-5.93339980523902));
#119651=CARTESIAN_POINT('Ctrl Pts',(17.4898526713405,21.7790594565463,-6.06057561192046));
#119652=CARTESIAN_POINT('Ctrl Pts',(20.2198982468525,21.6471728895478,-6.18775141860189));
#119653=CARTESIAN_POINT('Ctrl Pts',(21.5867244061235,19.2802489023316,-6.31492722528332));
#119654=CARTESIAN_POINT('Ctrl Pts',(20.3363529828215,16.8497933452978,-6.44210303196475));
#119655=CARTESIAN_POINT('Ctrl Pts',(17.615922151023,16.5855983409401,-6.56927883864619));
#119656=CARTESIAN_POINT('Ctrl Pts',(15.9212583499232,18.7300464079656,-6.69645464532763));
#119657=CARTESIAN_POINT('Ctrl Pts',(16.8071104343333,21.315739544336,-6.82363045200906));
#119658=CARTESIAN_POINT('Ctrl Pts',(19.4607640989881,21.9704647836472,-6.95080625869048));
#119659=CARTESIAN_POINT('Ctrl Pts',(21.4476568108886,20.0935523556623,-7.07798206537195));
#119660=CARTESIAN_POINT('Ctrl Pts',(20.9449378273356,17.4069529187342,-7.20515787205335));
#119661=CARTESIAN_POINT('Ctrl Pts',(18.4138206134801,16.3754547070776,-7.3323336787348));
#119662=CARTESIAN_POINT('Ctrl Pts',(16.1764481141826,17.9453933078879,-7.45950948541623));
#119663=CARTESIAN_POINT('Ctrl Pts',(16.2854707305501,20.6764474963007,-7.58668529209767));
#119664=CARTESIAN_POINT('Ctrl Pts',(18.640866978772,22.0630445627872,-7.7138610987791));
#119665=CARTESIAN_POINT('Ctrl Pts',(21.0817069934834,20.8330677607659,-7.84103690546054));
#119666=CARTESIAN_POINT('Ctrl Pts',(21.3686715568034,18.1149444651214,-7.96821271214196));
#119667=CARTESIAN_POINT('Ctrl Pts',(19.2384884929154,16.4023840938492,-8.09538851882341));
#119668=CARTESIAN_POINT('Ctrl Pts',(16.6454685488647,17.2665544941074,-8.22256432550483));
#119669=CARTESIAN_POINT('Ctrl Pts',(15.9685465823494,19.9146329601232,-8.34974013218628));
#119670=CARTESIAN_POINT('Ctrl Pts',(17.8287564831316,21.9171718576127,-8.47691593886771));
#119671=CARTESIAN_POINT('Ctrl Pts',(20.5194711248913,21.4369660397109,-8.60409174554914));
#119672=CARTESIAN_POINT('Ctrl Pts',(21.5721268283993,18.9145745394082,-8.73126755223057));
#119673=CARTESIAN_POINT('Ctrl Pts',(20.0209773208683,16.6641350009595,-8.858443358912));
#119674=CARTESIAN_POINT('Ctrl Pts',(17.2891060002617,16.7502860228609,-8.98561916559344));
#119675=CARTESIAN_POINT('Ctrl Pts',(15.8828352441794,19.0939893896534,-9.11279497227487));
#119676=CARTESIAN_POINT('Ctrl Pts',(17.0923311883199,21.5450427289413,-9.23997077895631));
#119677=CARTESIAN_POINT('Ctrl Pts',(19.8079563737189,21.8547567314554,-9.36714658563774));
#119678=CARTESIAN_POINT('Ctrl Pts',(21.5382932434809,19.7389880229077,-9.49432239231919));
#119679=CARTESIAN_POINT('Ctrl Pts',(20.6958651164175,17.1388230739748,-9.62149819900061));
#119680=CARTESIAN_POINT('Ctrl Pts',(18.0535475121228,16.439751840865,-9.74867400568204));
#119681=CARTESIAN_POINT('Ctrl Pts',(16.035502831811,18.2831287907025,-9.87584981236349));
#119682=CARTESIAN_POINT('Ctrl Pts',(16.4931618156892,20.9777699848882,-10.0030256190449));
#119683=CARTESIAN_POINT('Ctrl Pts',(19.0066507515693,22.0515093760514,-10.1302014257263));
#119684=CARTESIAN_POINT('Ctrl Pts',(21.2699995454986,20.5192577165824,-10.2573772324077));
#119685=CARTESIAN_POINT('Ctrl Pts',(21.2067261583164,17.7867608017806,-10.3845530390892));
#119686=CARTESIAN_POINT('Ctrl Pts',(18.874879995573,16.3609149530909,-10.5117288457706));
#119687=CARTESIAN_POINT('Ctrl Pts',(16.4137851808899,17.5498452387121,-10.6389046524521));
#119688=CARTESIAN_POINT('Ctrl Pts',(16.0813434539675,20.2627819149227,-10.7660804591335));
#119689=CARTESIAN_POINT('Ctrl Pts',(18.1825494655964,22.0107739651396,-10.8932562658149));
#119690=CARTESIAN_POINT('Ctrl Pts',(20.7896771156604,21.1901471759111,-11.0204320724963));
#119691=CARTESIAN_POINT('Ctrl Pts',(21.5108486018171,18.5537756925119,-11.1476078791778));
#119692=CARTESIAN_POINT('Ctrl Pts',(19.6844338464684,16.5203667192919,-11.2747836858592));
#119693=CARTESIAN_POINT('Ctrl Pts',(16.9860550275624,16.9554467815862,-11.4019594925407));
#119694=CARTESIAN_POINT('Ctrl Pts',(15.8913072311674,19.4598569263539,-11.5291352992221));
#119695=CARTESIAN_POINT('Ctrl Pts',(17.4045536127647,21.7359562869947,-11.6563111059035));
#119696=CARTESIAN_POINT('Ctrl Pts',(20.1374845399016,21.6955649707794,-11.783486912585));
#119697=CARTESIAN_POINT('Ctrl Pts',(21.5828055117534,19.3757395033677,-11.9106627192664));
#119698=CARTESIAN_POINT('Ctrl Pts',(20.4145242433828,16.9047757665027,-12.0378385259478));
#119699=CARTESIAN_POINT('Ctrl Pts',(17.7044662868062,16.5496296234525,-12.1650143326293));
#119700=CARTESIAN_POINT('Ctrl Pts',(15.9389416120162,18.6361256176097,-12.2921901393107));
#119701=CARTESIAN_POINT('Ctrl Pts',(16.7377095273126,21.2500331768819,-12.4193659459921));
#119702=CARTESIAN_POINT('Ctrl Pts',(19.3679500475393,21.9932543530368,-12.5465417526735));
#119703=CARTESIAN_POINT('Ctrl Pts',(21.416580746526,20.183929846461,-12.673717559355));
#119704=CARTESIAN_POINT('Ctrl Pts',(21.004110110314,17.4820025925939,-12.8008933660364));
#119705=CARTESIAN_POINT('Ctrl Pts',(18.5089543468127,16.3663231463401,-12.9280691727179));
#119706=CARTESIAN_POINT('Ctrl Pts',(16.2202640022022,17.8604581527614,-13.0552449793993));
#119707=CARTESIAN_POINT('Ctrl Pts',(16.2377704155193,20.5936314799435,-13.1824207860807));
#119708=CARTESIAN_POINT('Ctrl Pts',(18.5454125391162,22.0583262400653,-13.3095965927622));
#119709=CARTESIAN_POINT('Ctrl Pts',(21.0260719530159,20.9107758999245,-13.4367723994436));
#119710=CARTESIAN_POINT('Ctrl Pts',(21.4038976120531,18.2037866715935,-13.563948206125));
#119711=CARTESIAN_POINT('Ctrl Pts',(19.3322579245662,16.4208531573659,-13.6911240128065));
#119712=CARTESIAN_POINT('Ctrl Pts',(16.7117537233642,17.1977061952114,-13.8182998194879));
#119713=CARTESIAN_POINT('Ctrl Pts',(15.9465349662162,19.8216313398441,-13.9454756261693));
#119714=CARTESIAN_POINT('Ctrl Pts',(17.7386423679729,21.8853401302251,-14.0726514328508));
#119715=CARTESIAN_POINT('Ctrl Pts',(20.4439286182524,21.495507839393,-14.1998272395322));
#119716=CARTESIAN_POINT('Ctrl Pts',(21.5804614914246,19.0097813984656,-14.3270030462136));
#119717=CARTESIAN_POINT('Ctrl Pts',(20.1055426175397,16.708660535411,-14.4541788528951));
#119718=CARTESIAN_POINT('Ctrl Pts',(17.3723185195974,16.7032808184137,-14.5813546595765));
#119719=CARTESIAN_POINT('Ctrl Pts',(15.8883526644403,18.9985778039157,-14.708530466258));
#119720=CARTESIAN_POINT('Ctrl Pts',(17.0150916188663,21.4887589699166,-14.8357062729394));
#119721=CARTESIAN_POINT('Ctrl Pts',(19.7188223254962,21.8892376546847,-14.9628820796208));
#119722=CARTESIAN_POINT('Ctrl Pts',(21.5190396734505,19.8325995214557,-15.0900578863023));
#119723=CARTESIAN_POINT('Ctrl Pts',(20.7641559800708,17.2056824081085,-15.2172336929837));
#119724=CARTESIAN_POINT('Ctrl Pts',(18.1467301806671,16.4185197212751,-15.3444094996651));
#119725=CARTESIAN_POINT('Ctrl Pts',(16.0680879904256,18.1932843692987,-15.4715853063465));
#119726=CARTESIAN_POINT('Ctrl Pts',(16.4352546038082,20.9017399419349,-15.598761113028));
#119727=CARTESIAN_POINT('Ctrl Pts',(18.9113774419666,22.0590465570016,-15.7259369197094));
#119728=CARTESIAN_POINT('Ctrl Pts',(21.2247674864064,20.6034472257245,-15.8531127263909));
#119729=CARTESIAN_POINT('Ctrl Pts',(21.2530329565334,17.870363989867,-15.9802885330723));
#119730=CARTESIAN_POINT('Ctrl Pts',(18.9702420378592,16.3672310840514,-16.1074643397537));
#119731=CARTESIAN_POINT('Ctrl Pts',(16.4707137122836,17.4730796544138,-16.2346401464351));
#119732=CARTESIAN_POINT('Ctrl Pts',(16.0476100802981,20.1733622743496,-16.3618159531166));
#119733=CARTESIAN_POINT('Ctrl Pts',(18.0891024634763,21.9907372385088,-16.488991759798));
#119734=CARTESIAN_POINT('Ctrl Pts',(20.7222483095596,21.2578758162869,-16.6161675664795));
#119735=CARTESIAN_POINT('Ctrl Pts',(21.5312997362295,18.6471328760627,-16.7433433731609));
#119736=CARTESIAN_POINT('Ctrl Pts',(19.7740022749111,16.5537030245103,-16.8705191798423));
#119737=CARTESIAN_POINT('Ctrl Pts',(17.0625672761828,16.8981782175187,-16.9976949865238));
#119738=CARTESIAN_POINT('Ctrl Pts',(15.8845680607422,19.3645238460445,-17.1248707932052));
#119739=CARTESIAN_POINT('Ctrl Pts',(17.3207457938787,21.6900208745888,-17.2520465998866));
#119740=CARTESIAN_POINT('Ctrl Pts',(20.053496544683,21.7411701160866,-17.3792224065681));
#119741=CARTESIAN_POINT('Ctrl Pts',(21.5756911129322,19.4710453161425,-17.5063982132495));
#119742=CARTESIAN_POINT('Ctrl Pts',(20.4908104603086,16.9623450788714,-17.6335740199309));
#119743=CARTESIAN_POINT('Ctrl Pts',(17.794165250305,16.516646164469,-17.7607498266124));
#119744=CARTESIAN_POINT('Ctrl Pts',(15.959760090426,18.5428496637114,-17.8879256332938));
#119745=CARTESIAN_POINT('Ctrl Pts',(16.6705478588277,21.1820396264035,-18.0151014399752));
#119746=CARTESIAN_POINT('Ctrl Pts',(19.2744248944815,22.0129230684028,-18.1422772466567));
#119747=CARTESIAN_POINT('Ctrl Pts',(21.3824956319804,20.2732160020698,-18.2694530533381));
#119748=CARTESIAN_POINT('Ctrl Pts',(21.0607360113538,17.5589916824588,-18.3966288600195));
#119749=CARTESIAN_POINT('Ctrl Pts',(18.6043405137593,16.360382458875,-18.523804666701));
#119750=CARTESIAN_POINT('Ctrl Pts',(16.2668995473587,17.7770379002201,-18.6509804733824));
#119751=CARTESIAN_POINT('Ctrl Pts',(16.1928701204568,20.5092645659538,-18.7781562800638));
#119752=CARTESIAN_POINT('Ctrl Pts',(18.45016963826,22.0504140726478,-18.9053320867453));
#119753=CARTESIAN_POINT('Ctrl Pts',(20.9678658954356,20.9865773999889,-19.0325078934267));
#119754=CARTESIAN_POINT('Ctrl Pts',(21.4361288448778,18.2937586707072,-19.1596837001081));
#119755=CARTESIAN_POINT('Ctrl Pts',(19.4253562883709,16.4424519246523,-19.2868595067896));
#119756=CARTESIAN_POINT('Ctrl Pts',(16.780307255024,17.1311162137809,-19.414035313471));
#119757=CARTESIAN_POINT('Ctrl Pts',(15.9276500412235,19.7279447624144,-19.5412111201524));
#119758=CARTESIAN_POINT('Ctrl Pts',(17.6496447600855,21.8505086195232,-19.6683869268339));
#119759=CARTESIAN_POINT('Ctrl Pts',(20.3664680564733,21.5514870621786,-19.7955627335153));
#119760=CARTESIAN_POINT('Ctrl Pts',(21.5856033344346,19.1052140510933,-19.9227385401968));
#119761=CARTESIAN_POINT('Ctrl Pts',(20.1885693489379,16.7559927763657,-20.0499143468782));
#119762=CARTESIAN_POINT('Ctrl Pts',(17.457058641429,16.6590888438425,-20.1770901535596));
#119763=CARTESIAN_POINT('Ctrl Pts',(15.8970616522235,18.9034038719576,-20.3042659602411));
#119764=CARTESIAN_POINT('Ctrl Pts',(16.9397809084021,21.4299214440102,-20.4314417669225));
#119765=CARTESIAN_POINT('Ctrl Pts',(19.6285821382997,21.9207120974271,-20.5586175736039));
#119766=CARTESIAN_POINT('Ctrl Pts',(21.4966649457231,19.9255182070319,-20.6857933802854));
#119767=CARTESIAN_POINT('Ctrl Pts',(20.8301641839021,17.2747825617085,-20.8129691869668));
#119768=CARTESIAN_POINT('Ctrl Pts',(18.240582059696,16.40043638892,-20.9401449936482));
#119769=CARTESIAN_POINT('Ctrl Pts',(16.1036433297677,18.104549801285,-21.0673208003297));
#119770=CARTESIAN_POINT('Ctrl Pts',(16.3799647587305,20.8238745060694,-21.1944966070111));
#119771=CARTESIAN_POINT('Ctrl Pts',(18.8158302886401,22.0632713447717,-21.3216724136925));
#119772=CARTESIAN_POINT('Ctrl Pts',(21.176885810551,20.6863017024412,-21.4488482203739));
#119773=CARTESIAN_POINT('Ctrl Pts',(21.2962360890773,17.9550335586219,-21.5760240270554));
#119774=CARTESIAN_POINT('Ctrl Pts',(19.06587574408,16.377582661504,-21.7031998337368));
#119775=CARTESIAN_POINT('Ctrl Pts',(16.529138326029,17.396607333106,-21.8303756404183));
#119776=CARTESIAN_POINT('Ctrl Pts',(16.0189811762652,20.0863088421845,-21.9575514470997));
#119777=CARTESIAN_POINT('Ctrl Pts',(17.3340241117299,21.3345380991533,-22.0423353182207));
#119778=CARTESIAN_POINT('Ctrl Pts',(18.1101967966574,21.5422305581871,-22.0847272537811));
#119779=CARTESIAN_POINT('Ctrl Pts',(20.6946895702226,20.8620838326754,0.257713273515286));
#119780=CARTESIAN_POINT('Ctrl Pts',(21.2446793034262,20.2090078950207,0.21530268190311));
#119781=CARTESIAN_POINT('Ctrl Pts',(21.6307189736713,18.3216248822975,0.130500154730457));
#119782=CARTESIAN_POINT('Ctrl Pts',(19.54985825025,16.2898541338203,0.00330569199732501));
#119783=CARTESIAN_POINT('Ctrl Pts',(16.7212342529825,16.9459341572626,-0.12387011468411));
#119784=CARTESIAN_POINT('Ctrl Pts',(15.7390230172331,19.6762947228445,-0.251045921365544));
#119785=CARTESIAN_POINT('Ctrl Pts',(17.5046028706573,21.9817197183951,-0.378221728046978));
#119786=CARTESIAN_POINT('Ctrl Pts',(20.3980344048781,21.7441743961897,-0.505397534728411));
#119787=CARTESIAN_POINT('Ctrl Pts',(21.7648403718746,19.1831212459942,-0.632573341409846));
#119788=CARTESIAN_POINT('Ctrl Pts',(20.3510266276838,16.6473739692942,-0.75974914809128));
#119789=CARTESIAN_POINT('Ctrl Pts',(17.4536974328697,16.4637351954612,-0.886924954772716));
#119790=CARTESIAN_POINT('Ctrl Pts',(15.7309632043494,18.8004683182191,-1.01410076145415));
#119791=CARTESIAN_POINT('Ctrl Pts',(16.7633304940341,21.5138766926494,-1.14127656813558));
#119792=CARTESIAN_POINT('Ctrl Pts',(19.6036638866926,22.1145189554039,-1.26845237481702));
#119793=CARTESIAN_POINT('Ctrl Pts',(21.6461350846223,20.0513730033173,-1.39562818149845));
#119794=CARTESIAN_POINT('Ctrl Pts',(21.016902859507,17.2172316786593,-1.52280398817988));
#119795=CARTESIAN_POINT('Ctrl Pts',(18.2932490733073,16.2122517932659,-1.64997979486132));
#119796=CARTESIAN_POINT('Ctrl Pts',(15.9739568441929,17.9584358360373,-1.77715560154276));
#119797=CARTESIAN_POINT('Ctrl Pts',(16.1868329351487,20.853770497638,-1.90433140822419));
#119798=CARTESIAN_POINT('Ctrl Pts',(18.7365766963666,22.2419648047335,-2.03150721490562));
#119799=CARTESIAN_POINT('Ctrl Pts',(21.2839565072747,20.8494372260819,-2.15868302158706));
#119800=CARTESIAN_POINT('Ctrl Pts',(21.4919094864038,17.9537450817297,-2.28585882826849));
#119801=CARTESIAN_POINT('Ctrl Pts',(19.169651689263,16.2115063446496,-2.41303463494992));
#119802=CARTESIAN_POINT('Ctrl Pts',(16.4477105056032,17.2211168388571,-2.54021044163136));
#119803=CARTESIAN_POINT('Ctrl Pts',(15.8232980305526,20.0563216418289,-2.66738624831279));
#119804=CARTESIAN_POINT('Ctrl Pts',(17.8692739536042,22.1159962974782,-2.79456205499423));
#119805=CARTESIAN_POINT('Ctrl Pts',(20.7085823534422,21.5105171585006,-2.92173786167567));
#119806=CARTESIAN_POINT('Ctrl Pts',(21.7363340003116,18.7953737487032,-3.04891366835709));
#119807=CARTESIAN_POINT('Ctrl Pts',(20.0096305478046,16.4615416288479,-3.17608947503854));
#119808=CARTESIAN_POINT('Ctrl Pts',(17.1126152422242,16.6501669133465,-3.30326528171996));
#119809=CARTESIAN_POINT('Ctrl Pts',(15.7031198174278,19.1881976119062,-3.4304410884014));
#119810=CARTESIAN_POINT('Ctrl Pts',(17.0742688424951,21.7471480861189,-3.55761689508284));
#119811=CARTESIAN_POINT('Ctrl Pts',(19.9681181900429,21.9793401024969,-3.68479270176427));
#119812=CARTESIAN_POINT('Ctrl Pts',(21.7297406962381,19.671751897359,-3.8119685084457));
#119813=CARTESIAN_POINT('Ctrl Pts',(20.742957050273,16.9414524239027,-3.93914431512714));
#119814=CARTESIAN_POINT('Ctrl Pts',(17.9130800006189,16.2933219874959,-4.06632012180857));
#119815=CARTESIAN_POINT('Ctrl Pts',(15.8363460983557,18.3219800360464,-4.19349592849001));
#119816=CARTESIAN_POINT('Ctrl Pts',(16.4180298021666,21.1662587227194,-4.32067173517144));
#119817=CARTESIAN_POINT('Ctrl Pts',(19.1244724171678,22.2167088883417,-4.44784754185288));
#119818=CARTESIAN_POINT('Ctrl Pts',(21.4726808248689,20.5096077042429,-4.57502334853431));
#119819=CARTESIAN_POINT('Ctrl Pts',(21.3083195574551,17.6111145521858,-4.70219915521574));
#119820=CARTESIAN_POINT('Ctrl Pts',(18.7821798763678,16.1804169984081,-4.82937496189718));
#119821=CARTESIAN_POINT('Ctrl Pts',(16.2118381490933,17.5300912493964,-4.95655076857861));
#119822=CARTESIAN_POINT('Ctrl Pts',(15.9554233770066,20.4218949501003,-5.08372657526004));
#119823=CARTESIAN_POINT('Ctrl Pts',(18.2481801986013,22.2027776907038,-5.21090238194148));
#119824=CARTESIAN_POINT('Ctrl Pts',(20.9866465346018,21.238890090752,-5.33807818862291));
#119825=CARTESIAN_POINT('Ctrl Pts',(21.6584494901173,18.4145391975892,-5.46525399530435));
#119826=CARTESIAN_POINT('Ctrl Pts',(19.6472515502562,16.3208916567058,-5.59242980198579));
#119827=CARTESIAN_POINT('Ctrl Pts',(16.7982019958189,16.8787391404406,-5.71960560866721));
#119828=CARTESIAN_POINT('Ctrl Pts',(15.7251269610433,19.5762912063867,-5.84678141534867));
#119829=CARTESIAN_POINT('Ctrl Pts',(17.4125061877879,21.9387112630022,-5.97395722203007));
#119830=CARTESIAN_POINT('Ctrl Pts',(20.3122739660809,21.7986255366678,-6.10113302871153));
#119831=CARTESIAN_POINT('Ctrl Pts',(21.7640733392246,19.2845539865944,-6.22830883539295));
#119832=CARTESIAN_POINT('Ctrl Pts',(20.4359684911912,16.703001219096,-6.35548464207439));
#119833=CARTESIAN_POINT('Ctrl Pts',(17.5464131885679,16.422381669117,-6.48266044875582));
#119834=CARTESIAN_POINT('Ctrl Pts',(15.7463950754831,18.7001463565497,-6.60983625543726));
#119835=CARTESIAN_POINT('Ctrl Pts',(16.6873190489681,21.4465875546951,-6.7370120621187));
#119836=CARTESIAN_POINT('Ctrl Pts',(19.5059457636785,22.1420159276201,-6.86418786880012));
#119837=CARTESIAN_POINT('Ctrl Pts',(21.6163601525715,20.1484191063189,-6.99136367548156));
#119838=CARTESIAN_POINT('Ctrl Pts',(21.0823880009273,17.2947984377616,-7.118539482163));
#119839=CARTESIAN_POINT('Ctrl Pts',(18.3939156158299,16.1991737696759,-7.24571528884443));
#119840=CARTESIAN_POINT('Ctrl Pts',(16.0174495451912,17.8667127328943,-7.37289109552587));
#119841=CARTESIAN_POINT('Ctrl Pts',(16.1332499087027,20.7675518278046,-7.50006690220729));
#119842=CARTESIAN_POINT('Ctrl Pts',(18.6350770602241,22.2403512312061,-7.62724270888874));
#119843=CARTESIAN_POINT('Ctrl Pts',(21.2276598691396,20.9339089027185,-7.75441851557016));
#119844=CARTESIAN_POINT('Ctrl Pts',(21.5324645221063,18.0468045917732,-7.8815943222516));
#119845=CARTESIAN_POINT('Ctrl Pts',(19.2698516683375,16.2277773097598,-8.00877012893304));
#119846=CARTESIAN_POINT('Ctrl Pts',(16.5156281675744,17.1456716863595,-8.13594593561446));
#119847=CARTESIAN_POINT('Ctrl Pts',(15.7966231353776,19.9583766019922,-8.26312174229592));
#119848=CARTESIAN_POINT('Ctrl Pts',(17.7724790623024,22.0854098727205,-8.39029754897732));
#119849=CARTESIAN_POINT('Ctrl Pts',(20.6304707708447,21.5753504912249,-8.51747335565878));
#119850=CARTESIAN_POINT('Ctrl Pts',(21.7485682553881,18.8961462821721,-8.64464916234021));
#119851=CARTESIAN_POINT('Ctrl Pts',(20.1009864708203,16.5058008172007,-8.77182496902164));
#119852=CARTESIAN_POINT('Ctrl Pts',(17.199279444024,16.5973076988504,-8.89900077570308));
#119853=CARTESIAN_POINT('Ctrl Pts',(15.705583271835,19.0867150427652,-9.0261765823845));
#119854=CARTESIAN_POINT('Ctrl Pts',(16.9902714829968,21.6901461209486,-9.15335238906595));
#119855=CARTESIAN_POINT('Ctrl Pts',(19.8747223805114,22.0191145063235,-9.28052819574737));
#119856=CARTESIAN_POINT('Ctrl Pts',(21.7126312951226,19.7718121233893,-9.40770400242882));
#119857=CARTESIAN_POINT('Ctrl Pts',(20.8178308711669,17.0099994251714,-9.53487980911025));
#119858=CARTESIAN_POINT('Ctrl Pts',(18.011244960046,16.2674681448564,-9.66205561579168));
#119859=CARTESIAN_POINT('Ctrl Pts',(15.8677419388458,18.2254446454444,-9.78923142247312));
#119860=CARTESIAN_POINT('Ctrl Pts',(16.353852788716,21.0876070133732,-9.91640722915455));
#119861=CARTESIAN_POINT('Ctrl Pts',(19.0236009763425,22.2280989218993,-10.043583035836));
#119862=CARTESIAN_POINT('Ctrl Pts',(21.4276582428386,20.6005898318611,-10.1707588425174));
#119863=CARTESIAN_POINT('Ctrl Pts',(21.3604512588158,17.6982183187623,-10.2979346491988));
#119864=CARTESIAN_POINT('Ctrl Pts',(18.8836382607796,16.1837301043787,-10.4251104558803));
#119865=CARTESIAN_POINT('Ctrl Pts',(16.2695414460758,17.4465741256675,-10.5522862625617));
#119866=CARTESIAN_POINT('Ctrl Pts',(15.9164323930488,20.3281693740358,-10.6794620692432));
#119867=CARTESIAN_POINT('Ctrl Pts',(18.1482667414313,22.1848310610778,-10.8066378759246));
#119868=CARTESIAN_POINT('Ctrl Pts',(20.9174749998444,21.3131873263528,-10.933813682606));
#119869=CARTESIAN_POINT('Ctrl Pts',(21.6834804676428,18.5129171961597,-11.0609894892874));
#119870=CARTESIAN_POINT('Ctrl Pts',(19.7435206717827,16.3530947105848,-11.1881652959689));
#119871=CARTESIAN_POINT('Ctrl Pts',(16.8773883174812,16.8152229464412,-11.3153411026503));
#119872=CARTESIAN_POINT('Ctrl Pts',(15.7145819475737,19.4753279302437,-11.4425169093318));
#119873=CARTESIAN_POINT('Ctrl Pts',(17.3219042345475,21.8929284440893,-11.5696927160132));
#119874=CARTESIAN_POINT('Ctrl Pts',(20.2247367417761,21.8500260697353,-11.6968685226946));
#119875=CARTESIAN_POINT('Ctrl Pts',(21.7599108139823,19.3859810728298,-11.824044329376));
#119876=CARTESIAN_POINT('Ctrl Pts',(20.5189995235657,16.7614018021532,-11.9512201360575));
#119877=CARTESIAN_POINT('Ctrl Pts',(17.6404619598427,16.38417683879,-12.0783959427389));
#119878=CARTESIAN_POINT('Ctrl Pts',(15.7651776753385,18.6003866734043,-12.2055717494204));
#119879=CARTESIAN_POINT('Ctrl Pts',(16.6136036078165,21.3767963362328,-12.3327475561018));
#119880=CARTESIAN_POINT('Ctrl Pts',(19.4073616234801,22.1662222850487,-12.4599233627832));
#119881=CARTESIAN_POINT('Ctrl Pts',(21.5833521431366,20.2444152091134,-12.5870991694647));
#119882=CARTESIAN_POINT('Ctrl Pts',(21.1452389222041,17.3745138197983,-12.7142749761461));
#119883=CARTESIAN_POINT('Ctrl Pts',(18.4949636485153,16.1894745156307,-12.8414507828275));
#119884=CARTESIAN_POINT('Ctrl Pts',(16.0639893910444,17.7764973063501,-12.968626589509));
#119885=CARTESIAN_POINT('Ctrl Pts',(16.0825841477421,20.6795872832148,-13.0958023961904));
#119886=CARTESIAN_POINT('Ctrl Pts',(18.5336883834592,22.2353395785366,-13.2229782028718));
#119887=CARTESIAN_POINT('Ctrl Pts',(21.1685660946113,21.0164480222352,-13.3501540095533));
#119888=CARTESIAN_POINT('Ctrl Pts',(21.5698805201709,18.1411699642751,-13.4773298162347));
#119889=CARTESIAN_POINT('Ctrl Pts',(19.3694505830695,16.247394562952,-13.6045056229161));
#119890=CARTESIAN_POINT('Ctrl Pts',(16.5860341765131,17.072543208022,-13.7316814295976));
#119891=CARTESIAN_POINT('Ctrl Pts',(15.7732430952114,19.8595932321345,-13.858857236279));
#119892=CARTESIAN_POINT('Ctrl Pts',(17.6767627087548,22.0515992219996,-13.9860330429604));
#119893=CARTESIAN_POINT('Ctrl Pts',(20.5502319174689,21.6375317331515,-14.1132088496419));
#119894=CARTESIAN_POINT('Ctrl Pts',(21.7574210699713,18.9972719866817,-14.2403846563233));
#119895=CARTESIAN_POINT('Ctrl Pts',(20.1908090454502,16.5530944269748,-14.3675604630048));
#119896=CARTESIAN_POINT('Ctrl Pts',(17.2876651414952,16.5473802622938,-14.4947362696862));
#119897=CARTESIAN_POINT('Ctrl Pts',(15.7114437005529,18.9853718840723,-14.6219120763676));
#119898=CARTESIAN_POINT('Ctrl Pts',(16.9082300633519,21.6303632981543,-14.749087883049));
#119899=CARTESIAN_POINT('Ctrl Pts',(19.7800470229629,22.0557390488012,-14.8762636897305));
#119900=CARTESIAN_POINT('Ctrl Pts',(21.6921807640061,19.8712432865912,-15.0034394964119));
#119901=CARTESIAN_POINT('Ctrl Pts',(20.8903672594785,17.0810152882537,-15.1306153030934));
#119902=CARTESIAN_POINT('Ctrl Pts',(18.1102206336258,16.2449160611827,-15.2577911097748));
#119903=CARTESIAN_POINT('Ctrl Pts',(15.9023528603076,18.1300147520451,-15.3849669164562));
#119904=CARTESIAN_POINT('Ctrl Pts',(16.2923455858144,21.0068503143949,-15.5121427231376));
#119905=CARTESIAN_POINT('Ctrl Pts',(18.9224046901724,22.2361046763285,-15.6393185298191));
#119906=CARTESIAN_POINT('Ctrl Pts',(21.379614185011,20.6900132569022,-15.7664943365005));
#119907=CARTESIAN_POINT('Ctrl Pts',(21.4096368704371,17.7870189721836,-15.8936701431819));
#119908=CARTESIAN_POINT('Ctrl Pts',(18.9849287959905,16.1904388982563,-16.0208459498634));
#119909=CARTESIAN_POINT('Ctrl Pts',(16.33000912562,17.3650361580133,-16.1480217565448));
#119910=CARTESIAN_POINT('Ctrl Pts',(15.8806018739919,20.2331906693557,-16.2751975632263));
#119911=CARTESIAN_POINT('Ctrl Pts',(18.0490103011151,22.1635486858722,-16.4023733699077));
#119912=CARTESIAN_POINT('Ctrl Pts',(20.8458542617096,21.3851265389399,-16.5295491765891));
#119913=CARTESIAN_POINT('Ctrl Pts',(21.7052030136437,18.6120782340418,-16.6567249832706));
#119914=CARTESIAN_POINT('Ctrl Pts',(19.8386574142166,16.3885034761332,-16.783900789952));
#119915=CARTESIAN_POINT('Ctrl Pts',(16.9586572000173,16.754394094981,-16.9110765966334));
#119916=CARTESIAN_POINT('Ctrl Pts',(15.7074238146008,19.3740681575255,-17.0382524033149));
#119917=CARTESIAN_POINT('Ctrl Pts',(17.2328862287842,21.8441373066915,-17.1654282099963));
#119918=CARTESIAN_POINT('Ctrl Pts',(20.1355273584301,21.8984664079011,-17.2926040166777));
#119919=CARTESIAN_POINT('Ctrl Pts',(21.7523541253142,19.487211882838,-17.4197798233592));
#119920=CARTESIAN_POINT('Ctrl Pts',(20.6000283224083,16.8225500989152,-17.5469556300406));
#119921=CARTESIAN_POINT('Ctrl Pts',(17.7357373524709,16.3491428553155,-17.674131436722));
#119922=CARTESIAN_POINT('Ctrl Pts',(15.7872904024767,18.5013119150815,-17.8013072434035));
#119923=CARTESIAN_POINT('Ctrl Pts',(16.5422666147802,21.304575744541,-17.9284830500849));
#119924=CARTESIAN_POINT('Ctrl Pts',(19.3080221737182,22.1871137703668,-18.0556588567663));
#119925=CARTESIAN_POINT('Ctrl Pts',(21.5471480160826,20.3392521303006,-18.1828346634478));
#119926=CARTESIAN_POINT('Ctrl Pts',(21.2053851573897,17.4562891879729,-18.3100104701292));
#119927=CARTESIAN_POINT('Ctrl Pts',(18.5962798081749,16.1831645059201,-18.4371862768106));
#119928=CARTESIAN_POINT('Ctrl Pts',(16.1135241872327,17.6878909612598,-18.5643620834921));
#119929=CARTESIAN_POINT('Ctrl Pts',(16.0348924791393,20.5899754243741,-18.6915378901735));
#119930=CARTESIAN_POINT('Ctrl Pts',(18.4325243964945,22.226935525381,-18.8187136968549));
#119931=CARTESIAN_POINT('Ctrl Pts',(21.1067414672911,21.0969619702091,-18.9458895035364));
#119932=CARTESIAN_POINT('Ctrl Pts',(21.6041155128897,18.2367353666694,-19.0730653102178));
#119933=CARTESIAN_POINT('Ctrl Pts',(19.4683367108302,16.270336088174,-19.2002411168992));
#119934=CARTESIAN_POINT('Ctrl Pts',(16.6588495624458,17.0018134428338,-19.3274169235807));
#119935=CARTESIAN_POINT('Ctrl Pts',(15.7531841271558,19.760082322527,-19.4545927302621));
#119936=CARTESIAN_POINT('Ctrl Pts',(17.5822322738009,22.0146022966338,-19.5817685369435));
#119937=CARTESIAN_POINT('Ctrl Pts',(20.4679557667883,21.6969910872163,-19.708944343625));
#119938=CARTESIAN_POINT('Ctrl Pts',(21.7628825724515,19.0986375219567,-19.8361201503064));
#119939=CARTESIAN_POINT('Ctrl Pts',(20.2789974048699,16.6033692313319,-19.9632959569879));
#119940=CARTESIAN_POINT('Ctrl Pts',(17.3776734098626,16.5004409492398,-20.0904717636693));
#119941=CARTESIAN_POINT('Ctrl Pts',(15.7206941110155,18.8842811536826,-20.2176475703507));
#119942=CARTESIAN_POINT('Ctrl Pts',(16.8282374165171,21.5678679452165,-20.3448233770321));
#119943=CARTESIAN_POINT('Ctrl Pts',(19.6841967596975,22.0891702031096,-20.4719991837136));
#119944=CARTESIAN_POINT('Ctrl Pts',(21.668415038227,19.9699385658392,-20.5991749903951));
#119945=CARTESIAN_POINT('Ctrl Pts',(20.9604790789623,17.1544112786656,-20.7263507970764));
#119946=CARTESIAN_POINT('Ctrl Pts',(18.2099071213465,16.2257085193901,-20.8535266037579));
#119947=CARTESIAN_POINT('Ctrl Pts',(15.9401186134861,18.0357637096982,-20.9807024104393));
#119948=CARTESIAN_POINT('Ctrl Pts',(16.233618466875,20.9241441193076,-21.1078782171208));
#119949=CARTESIAN_POINT('Ctrl Pts',(18.8209175358886,22.2405921118336,-21.2350540238022));
#119950=CARTESIAN_POINT('Ctrl Pts',(21.3287557883375,20.7780186528654,-21.3622298304836));
#119951=CARTESIAN_POINT('Ctrl Pts',(21.4555258668686,17.8769523013118,-21.4894056371651));
#119952=CARTESIAN_POINT('Ctrl Pts',(19.0865078840121,16.2014340153418,-21.6165814438465));
#119953=CARTESIAN_POINT('Ctrl Pts',(16.3920658963632,17.2838096850018,-21.7437572505279));
#119954=CARTESIAN_POINT('Ctrl Pts',(15.8501931606037,20.1407252761597,-21.8709330572094));
#119955=CARTESIAN_POINT('Ctrl Pts',(17.2469900366476,21.4665547830909,-21.9557169283303));
#119956=CARTESIAN_POINT('Ctrl Pts',(18.0714160324376,21.6871591224115,-21.9981088638908));
#119957=CARTESIAN_POINT('Ctrl Pts',(20.3539256943887,20.5739122292573,4.33680868994202E-19));
#119958=CARTESIAN_POINT('Ctrl Pts',(20.4076089227952,20.5221116197655,8.86638463849601E-16));
#119959=CARTESIAN_POINT('Ctrl Pts',(20.4581355934374,20.4674384227593,2.54751254348717E-14));
#119960=CARTESIAN_POINT('Ctrl Pts',(20.5055119734051,20.410263943529,1.80931658544381E-15));
#119961=CARTESIAN_POINT('Ctrl Pts',(20.554575656102,20.3510532037209,-2.26993465278348E-14));
#119962=CARTESIAN_POINT('Ctrl Pts',(20.6002611628446,20.2891594084519,-2.64214052779902E-14));
#119963=CARTESIAN_POINT('Ctrl Pts',(20.6425471151747,20.2249453565124,-1.84539883374413E-14));
#119964=CARTESIAN_POINT('Ctrl Pts',(20.6826816163242,20.1639984273464,-1.08919426286634E-14));
#119965=CARTESIAN_POINT('Ctrl Pts',(20.7197537459369,20.1009604021273,8.86790207976305E-15));
#119966=CARTESIAN_POINT('Ctrl Pts',(20.753716758437,20.0361087206568,-9.26342336171615E-15));
#119967=CARTESIAN_POINT('Ctrl Pts',(20.7688150794711,20.0072787837823,-1.71121260304889E-14));
#119968=CARTESIAN_POINT('Ctrl Pts',(20.7832985639006,19.9780900549027,-2.84108754833378E-14));
#119969=CARTESIAN_POINT('Ctrl Pts',(20.7971611119739,19.9485653699547,-5.04457586814056E-15));
#119970=CARTESIAN_POINT('Ctrl Pts',(20.8039895160331,19.9340221216659,6.44146995798704E-15));
#119971=CARTESIAN_POINT('Ctrl Pts',(20.8106672398928,19.9193973462958,-1.4380597839645E-14));
#119972=CARTESIAN_POINT('Ctrl Pts',(20.8171934366481,19.9046937060787,-1.06165076729781E-14));
#119973=CARTESIAN_POINT('Ctrl Pts',(20.8232055554644,19.8911482928261,-7.43335609254726E-15));
#119974=CARTESIAN_POINT('Ctrl Pts',(20.8290895460591,19.8775345581707,-1.6413190692469E-15));
#119975=CARTESIAN_POINT('Ctrl Pts',(20.8348368052234,19.8638741231809,-4.3229309021342E-15));
#119976=CARTESIAN_POINT('Ctrl Pts',(20.8659056669685,19.7900277637341,-1.87793915734555E-14));
#119977=CARTESIAN_POINT('Ctrl Pts',(20.8930393190126,19.7146930410775,-3.51742239851522E-14));
#119978=CARTESIAN_POINT('Ctrl Pts',(20.9162161295942,19.6382510927703,-1.83048021185073E-14));
#119979=CARTESIAN_POINT('Ctrl Pts',(20.9398193031496,19.5604029105771,-1.1250486448073E-15));
#119980=CARTESIAN_POINT('Ctrl Pts',(20.9593192292438,19.4814055816641,-1.26531324379748E-14));
#119981=CARTESIAN_POINT('Ctrl Pts',(20.9746521650441,19.4016261052139,-4.85722573273506E-16));
#119982=CARTESIAN_POINT('Ctrl Pts',(20.9885844253231,19.3291345455208,1.05701850080071E-14));
#119983=CARTESIAN_POINT('Ctrl Pts',(20.9990759703875,19.2559962568409,-3.84562964731708E-15));
#119984=CARTESIAN_POINT('Ctrl Pts',(21.0060451898833,19.1824707413237,-1.37251321419285E-14));
#119985=CARTESIAN_POINT('Ctrl Pts',(21.0087031237876,19.1544294433498,-1.74137278270615E-14));
#119986=CARTESIAN_POINT('Ctrl Pts',(21.0108483731097,19.1263317159654,5.79109875787806E-15));
#119987=CARTESIAN_POINT('Ctrl Pts',(21.0124750503239,19.0981916687962,-1.26149091173033E-14));
#119988=CARTESIAN_POINT('Ctrl Pts',(21.0133685656744,19.0827346599387,-2.27851825805648E-14));
#119989=CARTESIAN_POINT('Ctrl Pts',(21.0141056048104,19.0672648807305,1.52001378915023E-15));
#119990=CARTESIAN_POINT('Ctrl Pts',(21.0146850898148,19.0517846622215,-5.00988139862102E-15));
#119991=CARTESIAN_POINT('Ctrl Pts',(21.0151328036157,19.0398245469222,-1.02380557977565E-14));
#119992=CARTESIAN_POINT('Ctrl Pts',(21.0154863000461,19.0278615000918,-2.2507103357516E-14));
#119993=CARTESIAN_POINT('Ctrl Pts',(21.015745158205,19.0159051388708,-1.89709359332824E-14));
#119994=CARTESIAN_POINT('Ctrl Pts',(21.017551908051,18.9324534374073,5.48211938410455E-15));
#119995=CARTESIAN_POINT('Ctrl Pts',(21.014756822678,18.8492079748144,1.85977283378329E-14));
#119996=CARTESIAN_POINT('Ctrl Pts',(21.0073036571099,18.7665493842094,1.59594559789866E-15));
#119997=CARTESIAN_POINT('Ctrl Pts',(20.9998648139147,18.6840496344554,-1.61673656061961E-14));
#119998=CARTESIAN_POINT('Ctrl Pts',(20.9877861501509,18.60213349936,-5.99635044273716E-15));
#119999=CARTESIAN_POINT('Ctrl Pts',(20.9709623839625,18.5211637972932,-8.99280649946377E-15));
#120000=CARTESIAN_POINT('Ctrl Pts',(20.9545246627898,18.4420520591064,-1.23431551296896E-14));
#120001=CARTESIAN_POINT('Ctrl Pts',(20.9335573250132,18.3638428657348,1.30025920795767E-14));
#120002=CARTESIAN_POINT('Ctrl Pts',(20.9083260331535,18.2867626991381,7.21644966006352E-16));
#120003=CARTESIAN_POINT('Ctrl Pts',(20.8979286030734,18.2549991395388,-4.46408057868302E-15));
#120004=CARTESIAN_POINT('Ctrl Pts',(20.886806477603,18.223427374722,-1.4774001875713E-14));
#120005=CARTESIAN_POINT('Ctrl Pts',(20.8749757625748,18.1920637286002,-7.46624984060418E-15));
#120006=CARTESIAN_POINT('Ctrl Pts',(20.868424493201,18.1746960805925,-3.19571242173869E-15));
#120007=CARTESIAN_POINT('Ctrl Pts',(20.8616536960862,18.1573871105346,-8.6285719324816E-15));
#120008=CARTESIAN_POINT('Ctrl Pts',(20.8546784987878,18.1401696684741,-5.19029264012261E-15));
#120009=CARTESIAN_POINT('Ctrl Pts',(20.8237193197693,18.06375062996,9.6487526525259E-15));
#120010=CARTESIAN_POINT('Ctrl Pts',(20.7887042347096,17.9890383341861,-9.83388335482747E-15));
#120011=CARTESIAN_POINT('Ctrl Pts',(20.7499612622237,17.916256394916,-1.42941214420489E-14));
#120012=CARTESIAN_POINT('Ctrl Pts',(20.7091543143746,17.8395971039635,-1.89919722093448E-14));
#120013=CARTESIAN_POINT('Ctrl Pts',(20.6642116622635,17.7650784733303,4.62724630464423E-15));
#120014=CARTESIAN_POINT('Ctrl Pts',(20.6154560962815,17.692967425201,-1.04916075827077E-14));
#120015=CARTESIAN_POINT('Ctrl Pts',(20.5667005302995,17.6208563770717,-2.56104614700597E-14));
#120016=CARTESIAN_POINT('Ctrl Pts',(20.5141314518022,17.55115202568,-2.07867077809236E-14));
#120017=CARTESIAN_POINT('Ctrl Pts',(20.4580183994378,17.484139989662,-2.21489493412719E-14));
#120018=CARTESIAN_POINT('Ctrl Pts',(20.4361046684505,17.457969897886,-2.30428670320704E-14));
#120019=CARTESIAN_POINT('Ctrl Pts',(20.4136499126721,17.4322106904206,-1.69753434272788E-15));
#120020=CARTESIAN_POINT('Ctrl Pts',(20.3906682863214,17.4068806089605,-9.07607322631065E-15));
#120021=CARTESIAN_POINT('Ctrl Pts',(20.3815365196799,17.3968156819022,-1.21213507505428E-14));
#120022=CARTESIAN_POINT('Ctrl Pts',(20.3723208008609,17.3868177123508,1.59343166306336E-14));
#120023=CARTESIAN_POINT('Ctrl Pts',(20.3630243250802,17.3768903879953,1.62925228863742E-14));
#120024=CARTESIAN_POINT('Ctrl Pts',(20.3025146980146,17.3122746444938,1.88054167317304E-14));
#120025=CARTESIAN_POINT('Ctrl Pts',(20.2387852814275,17.2508599884964,1.2995950010883E-14));
#120026=CARTESIAN_POINT('Ctrl Pts',(20.1721441631346,17.1929207844063,2.06223926824123E-14));
#120027=CARTESIAN_POINT('Ctrl Pts',(20.116951256814,17.1449348990317,2.69386962906269E-14));
#120028=CARTESIAN_POINT('Ctrl Pts',(20.0597599943144,17.0993329745171,-2.07314123176772E-15));
#120029=CARTESIAN_POINT('Ctrl Pts',(20.0007222400369,17.0562848434724,-1.36002320516582E-15));
#120030=CARTESIAN_POINT('Ctrl Pts',(19.9812253415778,17.0420684314475,-1.43164437014271E-15));
#120031=CARTESIAN_POINT('Ctrl Pts',(19.9615269094649,17.0281306668005,-7.66544549292576E-16));
#120032=CARTESIAN_POINT('Ctrl Pts',(19.9416319850871,17.0144780743264,-4.9960036108132E-15));
#120033=CARTESIAN_POINT('Ctrl Pts',(19.9257068710494,17.0035497044602,-8.18062758418038E-15));
#120034=CARTESIAN_POINT('Ctrl Pts',(19.9096544915251,16.9928033016912,-1.14146940178211E-14));
#120035=CARTESIAN_POINT('Ctrl Pts',(19.8934933769624,16.9822523936718,-9.88098491916389E-15));
#120036=CARTESIAN_POINT('Ctrl Pts',(19.8189655612139,16.9335963355889,-2.5256493517142E-15));
#120037=CARTESIAN_POINT('Ctrl Pts',(19.7420556121672,16.8890439678595,1.15006185245056E-14));
#120038=CARTESIAN_POINT('Ctrl Pts',(19.6630443965311,16.8488858958507,3.24740234702858E-15));
#120039=CARTESIAN_POINT('Ctrl Pts',(19.5852031544112,16.8093224720868,-5.05879407978434E-15));
#120040=CARTESIAN_POINT('Ctrl Pts',(19.5053217346575,16.774023445591,1.33716613157219E-14));
#120041=CARTESIAN_POINT('Ctrl Pts',(19.423636270734,16.7433040636654,-2.22044604925031E-16));
#120042=CARTESIAN_POINT('Ctrl Pts',(19.414941505442,16.7400342307853,-1.73426843035966E-15));
#120043=CARTESIAN_POINT('Ctrl Pts',(19.4062262753773,16.736816326208,-1.51681798593128E-14));
#120044=CARTESIAN_POINT('Ctrl Pts',(19.3974909960169,16.7336502196964,-9.99200722162641E-16));
#120045=CARTESIAN_POINT('Ctrl Pts',(18.071416109725,16.7348411664207,-0.001890963484983));
#120046=CARTESIAN_POINT('Ctrl Pts',(17.2469902101003,16.9554454800088,-0.0442828990454611));
#120047=CARTESIAN_POINT('Ctrl Pts',(15.8501940740727,18.2812783317349,-0.129066770166417));
#120048=CARTESIAN_POINT('Ctrl Pts',(16.3920656588252,21.1381881653492,-0.256242576847851));
#120049=CARTESIAN_POINT('Ctrl Pts',(19.0865079389648,22.2205670934987,-0.383418383529286));
#120050=CARTESIAN_POINT('Ctrl Pts',(21.4555257828913,20.5450469055032,-0.510594190210719));
#120051=CARTESIAN_POINT('Ctrl Pts',(21.3287556324384,17.643981848867,-0.637769996892156));
#120052=CARTESIAN_POINT('Ctrl Pts',(18.8209175760198,16.1814077573175,-0.764945803573588));
#120053=CARTESIAN_POINT('Ctrl Pts',(16.233618537572,17.4978560985894,-0.892121610255023));
#120054=CARTESIAN_POINT('Ctrl Pts',(15.9401187499945,20.386236157729,-1.01929741693645));
#120055=CARTESIAN_POINT('Ctrl Pts',(18.2099071291442,22.1962914055474,-1.14647322361789));
#120056=CARTESIAN_POINT('Ctrl Pts',(20.9604789958506,21.2675886098998,-1.27364903029932));
#120057=CARTESIAN_POINT('Ctrl Pts',(21.6684149124547,18.4520614803885,-1.40082483698076));
#120058=CARTESIAN_POINT('Ctrl Pts',(19.6841967236086,16.3328299069189,-1.52800064366219));
#120059=CARTESIAN_POINT('Ctrl Pts',(16.8282374931634,16.8541321563464,-1.65517645034363));
#120060=CARTESIAN_POINT('Ctrl Pts',(15.7206942359514,19.5377188303282,-1.78235225702506));
#120061=CARTESIAN_POINT('Ctrl Pts',(17.3776734650805,21.9215589406766,-1.9095280637065));
#120062=CARTESIAN_POINT('Ctrl Pts',(20.2789973416443,21.8186306606476,-2.03670387038792));
#120063=CARTESIAN_POINT('Ctrl Pts',(21.7628824476932,19.3233624738419,-2.16387967706936));
#120064=CARTESIAN_POINT('Ctrl Pts',(20.4679556955709,16.7250090148042,-2.29105548375079));
#120065=CARTESIAN_POINT('Ctrl Pts',(17.5822323211178,16.4073978188031,-2.41823129043223));
#120066=CARTESIAN_POINT('Ctrl Pts',(15.7531842497881,18.6619176999891,-2.54540709711366));
#120067=CARTESIAN_POINT('Ctrl Pts',(16.65884964778,21.4201864663384,-2.6725829037951));
#120068=CARTESIAN_POINT('Ctrl Pts',(19.468336680636,22.1516637908563,-2.79975871047653));
#120069=CARTESIAN_POINT('Ctrl Pts',(21.6041153948362,20.1852645932698,-2.92693451715797));
#120070=CARTESIAN_POINT('Ctrl Pts',(21.1067413697027,17.3250381073553,-3.0541103238394));
#120071=CARTESIAN_POINT('Ctrl Pts',(18.432524408893,16.1950645986679,-3.18128613052084));
#120072=CARTESIAN_POINT('Ctrl Pts',(16.0348925901549,17.8320246323415,-3.30846193720227));
#120073=CARTESIAN_POINT('Ctrl Pts',(16.1135242950128,20.7341089760952,-3.43563774388371));
#120074=CARTESIAN_POINT('Ctrl Pts',(18.5962798138393,22.2388353695441,-3.56281355056514));
#120075=CARTESIAN_POINT('Ctrl Pts',(21.2053850557409,20.9657107398561,-3.68998935724658));
#120076=CARTESIAN_POINT('Ctrl Pts',(21.5471479003775,18.0827479161047,-3.81716516392801));
#120077=CARTESIAN_POINT('Ctrl Pts',(19.3080221501088,16.2348863520412,-3.94434097060945));
#120078=CARTESIAN_POINT('Ctrl Pts',(16.5422667049268,17.1174243415679,-4.07151677729087));
#120079=CARTESIAN_POINT('Ctrl Pts',(15.7872905236753,19.9206880557286,-4.19869258397231));
#120080=CARTESIAN_POINT('Ctrl Pts',(17.7357373935294,22.0728570269757,-4.32586839065374));
#120081=CARTESIAN_POINT('Ctrl Pts',(20.6000282456582,21.5994498028477,-4.45304419733518));
#120082=CARTESIAN_POINT('Ctrl Pts',(21.7523540011689,18.9347881285228,-4.58022000401661));
#120083=CARTESIAN_POINT('Ctrl Pts',(20.1355273007852,16.5235337026348,-4.70739581069805));
#120084=CARTESIAN_POINT('Ctrl Pts',(17.2328862905255,16.5778628016098,-4.83457161737948));
#120085=CARTESIAN_POINT('Ctrl Pts',(15.7074239390844,19.0479318491813,-4.96174742406092));
#120086=CARTESIAN_POINT('Ctrl Pts',(16.9586572730372,21.6676058039782,-5.08892323074234));
#120087=CARTESIAN_POINT('Ctrl Pts',(19.8386573687817,22.0334964077772,-5.21609903742379));
#120088=CARTESIAN_POINT('Ctrl Pts',(21.7052028914376,19.8099217413247,-5.34327484410521));
#120089=CARTESIAN_POINT('Ctrl Pts',(20.8458541748489,17.0368735504825,-5.47045065078666));
#120090=CARTESIAN_POINT('Ctrl Pts',(18.0490103292891,16.2584514355665,-5.59762645746809));
#120091=CARTESIAN_POINT('Ctrl Pts',(15.8806019913527,18.188809372687,-5.72480226414952));
#120092=CARTESIAN_POINT('Ctrl Pts',(16.3300092244964,21.0569637660617,-5.85197807083096));
#120093=CARTESIAN_POINT('Ctrl Pts',(18.9849287856695,22.2315609775075,-5.97915387751239));
#120094=CARTESIAN_POINT('Ctrl Pts',(21.4096367603877,20.634980969248,-6.10632968419383));
#120095=CARTESIAN_POINT('Ctrl Pts',(21.3796140761966,17.73198680393,-6.23350549087526));
#120096=CARTESIAN_POINT('Ctrl Pts',(18.9224046824235,16.1858954480944,-6.36068129755669));
#120097=CARTESIAN_POINT('Ctrl Pts',(16.2923456862402,17.4151497594685,-6.48785710423813));
#120098=CARTESIAN_POINT('Ctrl Pts',(15.9023529767735,20.2919852034935,-6.61503291091956));
#120099=CARTESIAN_POINT('Ctrl Pts',(18.1102206592817,22.1770838168218,-6.742208717601));
#120100=CARTESIAN_POINT('Ctrl Pts',(20.8903671707866,21.3409846241399,-6.86938452428244));
#120101=CARTESIAN_POINT('Ctrl Pts',(21.6921806423356,18.550756740565,-6.99656033096386));
#120102=CARTESIAN_POINT('Ctrl Pts',(19.7800469799392,16.3662610682035,-7.1237361376453));
#120103=CARTESIAN_POINT('Ctrl Pts',(16.9082301384463,16.7916368013544,-7.25091194432673));
#120104=CARTESIAN_POINT('Ctrl Pts',(15.7114438248711,19.4366281066474,-7.37808775100818));
#120105=CARTESIAN_POINT('Ctrl Pts',(17.2876652009831,21.8746196281511,-7.50526355768959));
#120106=CARTESIAN_POINT('Ctrl Pts',(20.1908089855312,21.8689054637052,-7.63243936437104));
#120107=CARTESIAN_POINT('Ctrl Pts',(21.7574209456176,19.4247280045279,-7.75961517105247));
#120108=CARTESIAN_POINT('Ctrl Pts',(20.5502318427671,16.7844683666522,-7.88679097773391));
#120109=CARTESIAN_POINT('Ctrl Pts',(17.6767627522393,16.3704008948346,-8.01396678441534));
#120110=CARTESIAN_POINT('Ctrl Pts',(15.7732432169878,18.562406794542,-8.14114259109678));
#120111=CARTESIAN_POINT('Ctrl Pts',(16.5860342648591,21.3494567040227,-8.2683183977782));
#120112=CARTESIAN_POINT('Ctrl Pts',(19.3694505569332,22.1746053151545,-8.39549420445964));
#120113=CARTESIAN_POINT('Ctrl Pts',(21.5698804035306,20.2808299917227,-8.52267001114108));
#120114=CARTESIAN_POINT('Ctrl Pts',(21.1685659944773,17.4055520520233,-8.64984581782251));
#120115=CARTESIAN_POINT('Ctrl Pts',(18.5336883916982,16.1866605458549,-8.77702162450395));
#120116=CARTESIAN_POINT('Ctrl Pts',(16.0825842567954,17.7424127771882,-8.90419743118537));
#120117=CARTESIAN_POINT('Ctrl Pts',(16.0639895008622,20.6455026346484,-9.03137323786682));
#120118=CARTESIAN_POINT('Ctrl Pts',(18.4949636583467,22.2325253600934,-9.15854904454825));
#120119=CARTESIAN_POINT('Ctrl Pts',(21.1452388230294,21.0474861046668,-9.28572485122969));
#120120=CARTESIAN_POINT('Ctrl Pts',(21.5833520259422,18.1775848333912,-9.41290065791111));
#120121=CARTESIAN_POINT('Ctrl Pts',(19.4073615957849,16.2557778365002,-9.54007646459256));
#120122=CARTESIAN_POINT('Ctrl Pts',(16.6136036950289,17.0452037528466,-9.66725227127399));
#120123=CARTESIAN_POINT('Ctrl Pts',(15.7651777974467,19.8216133014809,-9.79442807795542));
#120124=CARTESIAN_POINT('Ctrl Pts',(17.6404620048199,22.0378230449422,-9.92160388463685));
#120125=CARTESIAN_POINT('Ctrl Pts',(20.5189994501482,21.6605980970946,-10.0487796913183));
#120126=CARTESIAN_POINT('Ctrl Pts',(21.7599106895262,19.0360189343673,-10.1759554979997));
#120127=CARTESIAN_POINT('Ctrl Pts',(20.2247366804621,16.5719740388084,-10.3031313046812));
#120128=CARTESIAN_POINT('Ctrl Pts',(17.3219042926274,16.5290716662188,-10.4303071113626));
#120129=CARTESIAN_POINT('Ctrl Pts',(15.7145820717629,18.9466720806279,-10.557482918044));
#120130=CARTESIAN_POINT('Ctrl Pts',(16.8773883938439,21.60677695502,-10.6846587247255));
#120131=CARTESIAN_POINT('Ctrl Pts',(19.7435206302607,22.0689051718692,-10.8118345314069));
#120132=CARTESIAN_POINT('Ctrl Pts',(21.6834803463302,19.9090827751282,-10.9390103380884));
#120133=CARTESIAN_POINT('Ctrl Pts',(20.9174749100379,17.1088127601106,-11.0661861447698));
#120134=CARTESIAN_POINT('Ctrl Pts',(18.1482667655227,16.2371690612364,-11.1933619514512));
#120135=CARTESIAN_POINT('Ctrl Pts',(15.9164325089359,18.0938306719134,-11.3205377581326));
#120136=CARTESIAN_POINT('Ctrl Pts',(16.2695415474392,20.9754258017613,-11.4477135648141));
#120137=CARTESIAN_POINT('Ctrl Pts',(18.8836382546247,22.2382697711092,-11.5748893714955));
#120138=CARTESIAN_POINT('Ctrl Pts',(21.3604511507894,20.7237816190169,-11.702065178177));
#120139=CARTESIAN_POINT('Ctrl Pts',(21.4276581320481,17.8214102252931,-11.8292409848584));
#120140=CARTESIAN_POINT('Ctrl Pts',(19.0236009644314,16.1939012021945,-11.9564167915398));
#120141=CARTESIAN_POINT('Ctrl Pts',(16.353852886612,17.3343930638118,-12.0835925982213));
#120142=CARTESIAN_POINT('Ctrl Pts',(15.8677420567354,20.1965553140193,-12.2107684049027));
#120143=CARTESIAN_POINT('Ctrl Pts',(18.0112449897728,22.1545317340756,-12.3379442115841));
#120144=CARTESIAN_POINT('Ctrl Pts',(20.8178307854584,21.4120004843013,-12.4651200182656));
#120145=CARTESIAN_POINT('Ctrl Pts',(21.712631172611,18.6501878996771,-12.592295824947));
#120146=CARTESIAN_POINT('Ctrl Pts',(19.8747223335935,16.4028856091748,-12.7194716316284));
#120147=CARTESIAN_POINT('Ctrl Pts',(16.9902715547168,16.731853981019,-12.8466474383099));
#120148=CARTESIAN_POINT('Ctrl Pts',(15.7055833963943,19.3352849521227,-12.9738232449913));
#120149=CARTESIAN_POINT('Ctrl Pts',(17.199279507147,21.824692193648,-13.1009990516727));
#120150=CARTESIAN_POINT('Ctrl Pts',(20.1009864145957,21.9161990715341,-13.2281748583542));
#120151=CARTESIAN_POINT('Ctrl Pts',(21.7485681313984,19.5258537048782,-13.3553506650356));
#120152=CARTESIAN_POINT('Ctrl Pts',(20.6304706928427,16.8466496060213,-13.482526471717));
#120153=CARTESIAN_POINT('Ctrl Pts',(17.77247910185,16.3365902455044,-13.6097022783985));
#120154=CARTESIAN_POINT('Ctrl Pts',(15.7966232561924,18.4636234287474,-13.7368780850799));
#120155=CARTESIAN_POINT('Ctrl Pts',(16.5156282588163,21.2763282286931,-13.8640538917614));
#120156=CARTESIAN_POINT('Ctrl Pts',(19.2698516462976,22.1942225675398,-13.9912296984428));
#120157=CARTESIAN_POINT('Ctrl Pts',(21.5324644070049,20.3751953603434,-14.1184055051242));
#120158=CARTESIAN_POINT('Ctrl Pts',(21.2276597665751,17.4880911681452,-14.2455813118056));
#120159=CARTESIAN_POINT('Ctrl Pts',(18.635077064293,16.1816488933915,-14.3727571184871));
#120160=CARTESIAN_POINT('Ctrl Pts',(16.1332500156721,17.6544482362164,-14.4999329251685));
#120161=CARTESIAN_POINT('Ctrl Pts',(16.0174496569233,20.5552872118146,-14.6271087318499));
#120162=CARTESIAN_POINT('Ctrl Pts',(18.3939156298174,22.2228261064472,-14.7542845385314));
#120163=CARTESIAN_POINT('Ctrl Pts',(21.0823879043376,21.1272014834248,-14.8814603452128));
#120164=CARTESIAN_POINT('Ctrl Pts',(21.6163600340196,18.2735809322375,-15.0086361518943));
#120165=CARTESIAN_POINT('Ctrl Pts',(19.5059457319285,16.279984192933,-15.1358119585757));
#120166=CARTESIAN_POINT('Ctrl Pts',(16.6873191331485,16.975412537255,-15.2629877652571));
#120167=CARTESIAN_POINT('Ctrl Pts',(15.7463951983637,19.7218536224386,-15.3901635719385));
#120168=CARTESIAN_POINT('Ctrl Pts',(17.5464132374134,21.9996182161866,-15.51733937862));
#120169=CARTESIAN_POINT('Ctrl Pts',(20.4359684211888,21.7189986777498,-15.6445151853014));
#120170=CARTESIAN_POINT('Ctrl Pts',(21.7640732145973,19.137446016431,-15.7716909919829));
#120171=CARTESIAN_POINT('Ctrl Pts',(20.3122739011664,16.6233745697617,-15.8988667986643));
#120172=CARTESIAN_POINT('Ctrl Pts',(17.4125062421414,16.4832888491888,-16.0260426053457));
#120173=CARTESIAN_POINT('Ctrl Pts',(15.7251270847987,18.8457088086375,-16.1532184120272));
#120174=CARTESIAN_POINT('Ctrl Pts',(16.7982020754384,21.543260763633,-16.2803942187086));
#120175=CARTESIAN_POINT('Ctrl Pts',(19.6472515126938,22.1011082244237,-16.40757002539));
#120176=CARTESIAN_POINT('Ctrl Pts',(21.6584493698341,20.0074607696524,-16.5347458320715));
#120177=CARTESIAN_POINT('Ctrl Pts',(20.9866464419503,17.1831099926555,-16.6619216387529));
#120178=CARTESIAN_POINT('Ctrl Pts',(18.2481802185833,16.2192224323484,-16.7890974454343));
#120179=CARTESIAN_POINT('Ctrl Pts',(15.9554234912899,18.0001050997038,-16.9162732521158));
#120180=CARTESIAN_POINT('Ctrl Pts',(16.2118382528302,20.8919086814673,-17.0434490587972));
#120181=CARTESIAN_POINT('Ctrl Pts',(18.782179874386,22.2415828769435,-17.1706248654786));
#120182=CARTESIAN_POINT('Ctrl Pts',(21.3083194515728,20.8108853820109,-17.2978006721601));
#120183=CARTESIAN_POINT('Ctrl Pts',(21.4726807122266,17.9123923491693,-17.4249764788415));
#120184=CARTESIAN_POINT('Ctrl Pts',(19.1244724011078,16.2052912352836,-17.552152285523));
#120185=CARTESIAN_POINT('Ctrl Pts',(16.418029897423,17.2557413577005,-17.6793280922044));
#120186=CARTESIAN_POINT('Ctrl Pts',(15.8363462175366,20.1000199273879,-17.8065038988858));
#120187=CARTESIAN_POINT('Ctrl Pts',(17.9130800343833,22.1286778924994,-17.9336797055672));
#120188=CARTESIAN_POINT('Ctrl Pts',(20.7429569676441,21.4805474827506,-18.0608555122487));
#120189=CARTESIAN_POINT('Ctrl Pts',(21.7297405730228,18.7502481215919,-18.1880313189301));
#120190=CARTESIAN_POINT('Ctrl Pts',(19.9681181392836,16.4426600113656,-18.3152071256115));
#120191=CARTESIAN_POINT('Ctrl Pts',(17.0742689107603,16.6748520181929,-18.442382932293));
#120192=CARTESIAN_POINT('Ctrl Pts',(15.7031199420884,19.2338023871561,-18.5695587389744));
#120193=CARTESIAN_POINT('Ctrl Pts',(17.1126153089119,21.7718329813254,-18.6967345456558));
#120194=CARTESIAN_POINT('Ctrl Pts',(20.0096304953375,21.9604582580674,-18.8239103523373));
#120195=CARTESIAN_POINT('Ctrl Pts',(21.7363338768253,19.6266262342004,-18.9510861590187));
#120196=CARTESIAN_POINT('Ctrl Pts',(20.708582272227,16.9114829360825,-19.0782619657001));
#120197=CARTESIAN_POINT('Ctrl Pts',(17.8692739891718,16.3060038219983,-19.2054377723816));
#120198=CARTESIAN_POINT('Ctrl Pts',(15.8232981502683,18.3656783929507,-19.332613579063));
#120199=CARTESIAN_POINT('Ctrl Pts',(16.4477105996423,21.2008830792771,-19.4597893857445));
#120200=CARTESIAN_POINT('Ctrl Pts',(19.1696516713374,22.2104935320204,-19.5869651924259));
#120201=CARTESIAN_POINT('Ctrl Pts',(21.4919093729839,20.4682548664865,-19.7141409991073));
#120202=CARTESIAN_POINT('Ctrl Pts',(21.2839564023691,17.5725628414412,-19.8413168057888));
#120203=CARTESIAN_POINT('Ctrl Pts',(18.7365766963097,16.1800353196856,-19.9684926124702));
#120204=CARTESIAN_POINT('Ctrl Pts',(16.186833039821,17.5682295703764,-20.0956684191516));
#120205=CARTESIAN_POINT('Ctrl Pts',(15.9739569578914,20.4635641116309,-20.222844225833));
#120206=CARTESIAN_POINT('Ctrl Pts',(18.2932490910976,22.2097480848697,-20.3500200325145));
#120207=CARTESIAN_POINT('Ctrl Pts',(21.0169027662538,21.2047682366741,-20.4771958391959));
#120208=CARTESIAN_POINT('Ctrl Pts',(21.6461349636216,18.3706270360342,-20.6043716458773));
#120209=CARTESIAN_POINT('Ctrl Pts',(19.6036638532537,16.3074811554586,-20.7315474525588));
#120210=CARTESIAN_POINT('Ctrl Pts',(16.7633305706532,16.9081234172833,-20.8587232592402));
#120211=CARTESIAN_POINT('Ctrl Pts',(15.7309633363042,19.6215316380409,-20.9858990659217));
#120212=CARTESIAN_POINT('Ctrl Pts',(17.4536974694716,21.9582647385426,-21.1130748726031));
#120213=CARTESIAN_POINT('Ctrl Pts',(20.3510265917206,21.7746258438458,-21.2402506792845));
#120214=CARTESIAN_POINT('Ctrl Pts',(21.7648401891172,19.2388788921253,-21.367426485966));
#120215=CARTESIAN_POINT('Ctrl Pts',(20.3980344469297,16.677825473566,-21.4946022926474));
#120216=CARTESIAN_POINT('Ctrl Pts',(17.5046027110691,16.4402807821758,-21.6217780993288));
#120217=CARTESIAN_POINT('Ctrl Pts',(15.7390235403886,18.7457046750729,-21.7489539060103));
#120218=CARTESIAN_POINT('Ctrl Pts',(16.7212335728181,21.4760667201902,-21.8761297126917));
#120219=CARTESIAN_POINT('Ctrl Pts',(19.5498596762323,22.1321442401452,-22.0033055193731));
#120220=CARTESIAN_POINT('Ctrl Pts',(21.6307161859342,20.100377524994,-22.1304999838292));
#120221=CARTESIAN_POINT('Ctrl Pts',(21.2446789959721,18.2129921435845,-22.2153025127247));
#120222=CARTESIAN_POINT('Ctrl Pts',(20.6946892744878,17.5599162803241,-22.2577131060598));
#120223=CARTESIAN_POINT('Ctrl Pts',(18.1101968784744,16.8797697475724,0.0847274365222686));
#120224=CARTESIAN_POINT('Ctrl Pts',(17.3340242953481,17.0874621793657,0.0423355009617904));
#120225=CARTESIAN_POINT('Ctrl Pts',(16.0189820756719,18.3356945672447,-0.0424483701591659));
#120226=CARTESIAN_POINT('Ctrl Pts',(16.5291381343926,21.0253906167311,-0.1696241768406));
#120227=CARTESIAN_POINT('Ctrl Pts',(19.065875791,22.0444183413159,-0.296799983522035));
#120228=CARTESIAN_POINT('Ctrl Pts',(21.2962359728301,20.4669656763903,-0.423975790203469));
#120229=CARTESIAN_POINT('Ctrl Pts',(21.1768856283234,17.7356987913358,-0.551151596884904));
#120230=CARTESIAN_POINT('Ctrl Pts',(18.8158303252349,16.3587285734324,-0.678327403566337));
#120231=CARTESIAN_POINT('Ctrl Pts',(16.3799648594531,17.5981257224815,-0.805503210247772));
#120232=CARTESIAN_POINT('Ctrl Pts',(16.1036434964602,20.3174500578439,-0.932679016929205));
#120233=CARTESIAN_POINT('Ctrl Pts',(18.2405820741981,22.0215634996219,-1.05985482361064));
#120234=CARTESIAN_POINT('Ctrl Pts',(20.8301640752336,21.1472173052792,-1.18703063029207));
#120235=CARTESIAN_POINT('Ctrl Pts',(21.4966647872182,18.4964818468598,-1.31420643697351));
#120236=CARTESIAN_POINT('Ctrl Pts',(19.6285820913403,16.501288045487,-1.44138224365494));
#120237=CARTESIAN_POINT('Ctrl Pts',(16.9397810066015,16.992078683811,-1.56855805033638));
#120238=CARTESIAN_POINT('Ctrl Pts',(15.8970618110187,19.518596108525,-1.69573385701782));
#120239=CARTESIAN_POINT('Ctrl Pts',(17.4570587119471,21.7629110154817,-1.82290966369925));
#120240=CARTESIAN_POINT('Ctrl Pts',(20.1885692683029,21.6660070863072,-1.95008547038068));
#120241=CARTESIAN_POINT('Ctrl Pts',(21.5856031755938,19.3167859434159,-2.07726127706212));
#120242=CARTESIAN_POINT('Ctrl Pts',(20.3664679657325,16.8705130678377,-2.20443708374355));
#120243=CARTESIAN_POINT('Ctrl Pts',(17.64964482037,16.5714915274638,-2.33161289042498));
#120244=CARTESIAN_POINT('Ctrl Pts',(15.927650197406,18.6940552662862,-2.45878869710642));
#120245=CARTESIAN_POINT('Ctrl Pts',(16.780307363717,21.2908836705225,-2.58596450378785));
#120246=CARTESIAN_POINT('Ctrl Pts',(19.4253562499103,21.979547921279,-2.71314031046929));
#120247=CARTESIAN_POINT('Ctrl Pts',(21.4361286945186,20.128241278265,-2.84031611715073));
#120248=CARTESIAN_POINT('Ctrl Pts',(20.9678657711395,17.4354226988042,-2.96749192383215));
#120249=CARTESIAN_POINT('Ctrl Pts',(18.4501696540519,16.3715860853484,-3.0946677305136));
#120250=CARTESIAN_POINT('Ctrl Pts',(16.1928702618537,17.9127355062838,-3.22184353719502));
#120251=CARTESIAN_POINT('Ctrl Pts',(16.2668996846349,20.6449620199907,-3.34901934387646));
#120252=CARTESIAN_POINT('Ctrl Pts',(18.6043405209739,22.0616173825078,-3.47619515055789));
#120253=CARTESIAN_POINT('Ctrl Pts',(21.0607358818871,20.8630082256189,-3.60337095723933));
#120254=CARTESIAN_POINT('Ctrl Pts',(21.3824954846104,18.1487840570351,-3.73054676392076));
#120255=CARTESIAN_POINT('Ctrl Pts',(19.2744248644109,16.4090770875045,-3.8577225706022));
#120256=CARTESIAN_POINT('Ctrl Pts',(16.6705479736445,17.2399604832709,-3.98489837728363));
#120257=CARTESIAN_POINT('Ctrl Pts',(15.9597602447928,19.8791502991104,-4.11207418396507));
#120258=CARTESIAN_POINT('Ctrl Pts',(17.7941653025999,21.9053536856092,-4.23924999064649));
#120259=CARTESIAN_POINT('Ctrl Pts',(20.4908103625543,21.4596547960069,-4.36642579732794));
#120260=CARTESIAN_POINT('Ctrl Pts',(21.5756909548122,18.9509546983274,-4.49360160400936));
#120261=CARTESIAN_POINT('Ctrl Pts',(20.0534964712626,16.6808300246996,-4.62077741069081));
#120262=CARTESIAN_POINT('Ctrl Pts',(17.3207458725165,16.7319792633511,-4.74795321737223));
#120263=CARTESIAN_POINT('Ctrl Pts',(15.8845682192929,19.0574761624978,-4.87512902405368));
#120264=CARTESIAN_POINT('Ctrl Pts',(17.062567369186,21.5238216537891,-5.0023048307351));
#120265=CARTESIAN_POINT('Ctrl Pts',(19.7740022170421,21.86829682763,-5.12948063741654));
#120266=CARTESIAN_POINT('Ctrl Pts',(21.5312995805795,19.7748670925622,-5.25665644409798));
#120267=CARTESIAN_POINT('Ctrl Pts',(20.7222481989278,17.1641242976074,-5.3838322507794));
#120268=CARTESIAN_POINT('Ctrl Pts',(18.0891024993605,16.4312629161638,-5.51100805746085));
#120269=CARTESIAN_POINT('Ctrl Pts',(16.0476102297768,18.2486377791988,-5.63818386414227));
#120270=CARTESIAN_POINT('Ctrl Pts',(16.4707138382194,20.948920248883,-5.76535967082371));
#120271=CARTESIAN_POINT('Ctrl Pts',(18.9702420247138,22.0547687577129,-5.89253547750515));
#120272=CARTESIAN_POINT('Ctrl Pts',(21.253032816367,20.5516359355363,-6.01971128418657));
#120273=CARTESIAN_POINT('Ctrl Pts',(21.2247673478128,17.8185528517555,-6.14688709086802));
#120274=CARTESIAN_POINT('Ctrl Pts',(18.911377432097,16.3629536014721,-6.27406289754945));
#120275=CARTESIAN_POINT('Ctrl Pts',(16.4352547317172,17.5202601521426,-6.40123870423088));
#120276=CARTESIAN_POINT('Ctrl Pts',(16.0680881387646,20.2287155740725,-6.52841451091232));
#120277=CARTESIAN_POINT('Ctrl Pts',(18.1467302133443,22.003480123343,-6.65559031759375));
#120278=CARTESIAN_POINT('Ctrl Pts',(20.7641558671069,21.2163174803099,-6.78276612427519));
#120279=CARTESIAN_POINT('Ctrl Pts',(21.5190395184827,18.5894005131322,-6.90994193095662));
#120280=CARTESIAN_POINT('Ctrl Pts',(19.718822270698,16.5327624943404,-7.03711773763806));
#120281=CARTESIAN_POINT('Ctrl Pts',(17.0150917145117,16.9332411568245,-7.16429354431949));
#120282=CARTESIAN_POINT('Ctrl Pts',(15.8883528227805,19.4234221842643,-7.29146935100092));
#120283=CARTESIAN_POINT('Ctrl Pts',(17.3723185953652,21.7187190420494,-7.41864515768236));
#120284=CARTESIAN_POINT('Ctrl Pts',(20.1055425412228,21.7133393253515,-7.54582096436379));
#120285=CARTESIAN_POINT('Ctrl Pts',(21.5804613330392,19.4122185903382,-7.67299677104523));
#120286=CARTESIAN_POINT('Ctrl Pts',(20.4439285231071,16.9264922877238,-7.80017257772666));
#120287=CARTESIAN_POINT('Ctrl Pts',(17.7386424233578,16.5366600185829,-7.9273483844081));
#120288=CARTESIAN_POINT('Ctrl Pts',(15.946535121319,18.600368694133,-8.05452419108952));
#120289=CARTESIAN_POINT('Ctrl Pts',(16.7117538358879,21.2242936927628,-8.18169999777097));
#120290=CARTESIAN_POINT('Ctrl Pts',(19.3322578912771,22.0011466873821,-8.30887580445239));
#120291=CARTESIAN_POINT('Ctrl Pts',(21.4038974634922,20.2182132723624,-8.43605161113384));
#120292=CARTESIAN_POINT('Ctrl Pts',(21.0260718254785,17.5112241946562,-8.56322741781526));
#120293=CARTESIAN_POINT('Ctrl Pts',(18.5454125496099,16.3636739183683,-8.69040322449671));
#120294=CARTESIAN_POINT('Ctrl Pts',(16.237770554417,17.82836859699,-8.81757903117813));
#120295=CARTESIAN_POINT('Ctrl Pts',(16.2202641420738,20.5615417720903,-8.94475483785957));
#120296=CARTESIAN_POINT('Ctrl Pts',(18.5089543593347,22.0556766953737,-9.071930644541));
#120297=CARTESIAN_POINT('Ctrl Pts',(21.0041099839982,20.9399973111998,-9.19910645122244));
#120298=CARTESIAN_POINT('Ctrl Pts',(21.4165805972594,18.2380702076759,-9.32628225790388));
#120299=CARTESIAN_POINT('Ctrl Pts',(19.3679500122646,16.4287458017761,-9.4534580645853));
#120300=CARTESIAN_POINT('Ctrl Pts',(16.7377096383923,17.1719669365758,-9.58063387126675));
#120301=CARTESIAN_POINT('Ctrl Pts',(15.9389417675414,19.7858743504024,-9.70780967794817));
#120302=CARTESIAN_POINT('Ctrl Pts',(17.7044663440924,21.8723702284609,-9.83498548462961));
#120303=CARTESIAN_POINT('Ctrl Pts',(20.4145241498733,21.5172241051723,-9.96216129131105));
#120304=CARTESIAN_POINT('Ctrl Pts',(21.5828053532376,19.0462605057991,-10.0893370979925));
#120305=CARTESIAN_POINT('Ctrl Pts',(20.1374844618078,16.7264351674692,-10.2165129046739));
#120306=CARTESIAN_POINT('Ctrl Pts',(17.4045536867392,16.6860438535011,-10.3436887113554));
#120307=CARTESIAN_POINT('Ctrl Pts',(15.8913073893432,18.9621430874931,-10.4708645180368));
#120308=CARTESIAN_POINT('Ctrl Pts',(16.986055124823,21.4665530929081,-10.5980403247182));
#120309=CARTESIAN_POINT('Ctrl Pts',(19.6844337935833,21.9016331309934,-10.7252161313997));
#120310=CARTESIAN_POINT('Ctrl Pts',(21.5108484473051,19.8682242709185,-10.8523919380811));
#120311=CARTESIAN_POINT('Ctrl Pts',(20.7896770012766,17.2318529342145,-10.9795677447625));
#120312=CARTESIAN_POINT('Ctrl Pts',(18.182549496281,16.4112261906481,-11.106743551444));
#120313=CARTESIAN_POINT('Ctrl Pts',(16.0813436015692,18.1592181436015,-11.2339193581254));
#120314=CARTESIAN_POINT('Ctrl Pts',(16.4137853099934,20.8721546688561,-11.3610951648069));
#120315=CARTESIAN_POINT('Ctrl Pts',(18.8748799877338,22.0610848883219,-11.4882709714883));
#120316=CARTESIAN_POINT('Ctrl Pts',(21.2067260207266,20.6352391189707,-11.6154467781697));
#120317=CARTESIAN_POINT('Ctrl Pts',(21.2699994043883,17.902742356213,-11.7426225848512));
#120318=CARTESIAN_POINT('Ctrl Pts',(19.0066507363984,16.3704907820029,-11.8697983915326));
#120319=CARTESIAN_POINT('Ctrl Pts',(16.4931619403762,17.4442301134199,-11.996974198214));
#120320=CARTESIAN_POINT('Ctrl Pts',(16.0355029819632,20.1388711576679,-12.1241500048955));
#120321=CARTESIAN_POINT('Ctrl Pts',(18.053547549985,21.9822480049345,-12.2513258115769));
#120322=CARTESIAN_POINT('Ctrl Pts',(20.6958650072534,21.2831768107233,-12.3785016182583));
#120323=CARTESIAN_POINT('Ctrl Pts',(21.5382930874419,18.6830120064713,-12.5056774249398));
#120324=CARTESIAN_POINT('Ctrl Pts',(19.807956313961,16.5672434156512,-12.6328532316212));
#120325=CARTESIAN_POINT('Ctrl Pts',(17.0923312796673,16.8769574009315,-12.7600290383026));
#120326=CARTESIAN_POINT('Ctrl Pts',(15.8828354028266,19.3280106038356,-12.8872048449841));
#120327=CARTESIAN_POINT('Ctrl Pts',(17.2891060806598,21.6717138402177,-13.0143806516655));
#120328=CARTESIAN_POINT('Ctrl Pts',(20.0209772492569,21.7578648573255,-13.1415564583469));
#120329=CARTESIAN_POINT('Ctrl Pts',(21.5721266704775,19.507425444098,-13.2687322650284));
#120330=CARTESIAN_POINT('Ctrl Pts',(20.5194710255427,16.9850340841485,-13.3959080717098));
#120331=CARTESIAN_POINT('Ctrl Pts',(17.8287565335022,16.5048282929666,-13.5230838783912));
#120332=CARTESIAN_POINT('Ctrl Pts',(15.9685467362274,18.5073670790289,-13.6502596850727));
#120333=CARTESIAN_POINT('Ctrl Pts',(16.6454686650766,21.1554453976977,-13.7774354917541));
#120334=CARTESIAN_POINT('Ctrl Pts',(19.2384884648439,22.0196157498711,-13.9046112984355));
#120335=CARTESIAN_POINT('Ctrl Pts',(21.3686714102025,20.3070554738911,-14.031787105117));
#120336=CARTESIAN_POINT('Ctrl Pts',(21.0817068628502,17.5889323294909,-14.1589629117984));
#120337=CARTESIAN_POINT('Ctrl Pts',(18.6408669839544,16.3589555959089,-14.2861387184799));
#120338=CARTESIAN_POINT('Ctrl Pts',(16.2854708667935,17.7455525852409,-14.4133145251613));
#120339=CARTESIAN_POINT('Ctrl Pts',(16.1764482564922,20.4766066216898,-14.5404903318427));
#120340=CARTESIAN_POINT('Ctrl Pts',(18.4138206312956,22.0465451351444,-14.6676661385241));
#120341=CARTESIAN_POINT('Ctrl Pts',(20.9449377043124,21.0150469808834,-14.7948419452056));
#120342=CARTESIAN_POINT('Ctrl Pts',(21.4476566598927,18.3284476934456,-14.922017751887));
#120343=CARTESIAN_POINT('Ctrl Pts',(19.4607640585489,16.4515353698976,-15.0491935585684));
#120344=CARTESIAN_POINT('Ctrl Pts',(16.8071105415512,17.1062605727777,-15.1763693652499));
#120345=CARTESIAN_POINT('Ctrl Pts',(15.9212585064325,19.6919535652726,-15.3035451719313));
#120346=CARTESIAN_POINT('Ctrl Pts',(17.615922213236,21.8364015129747,-15.4307209786127));
#120347=CARTESIAN_POINT('Ctrl Pts',(20.3363528936617,21.5722065233178,-15.5578967852942));
#120348=CARTESIAN_POINT('Ctrl Pts',(21.5867242473895,19.1417511015219,-15.6850725919756));
#120349=CARTESIAN_POINT('Ctrl Pts',(20.2198981641729,16.7748272460081,-15.8122483986571));
#120350=CARTESIAN_POINT('Ctrl Pts',(17.4898527405687,16.642940686348,-15.9394242053385));
#120351=CARTESIAN_POINT('Ctrl Pts',(15.9012352070049,18.8670891552265,-16.0666000120199));
#120352=CARTESIAN_POINT('Ctrl Pts',(16.9115035498021,21.4067544786704,-16.1937758187014));
#120353=CARTESIAN_POINT('Ctrl Pts',(19.5937992687688,21.931951351827,-16.3209516253828));
#120354=CARTESIAN_POINT('Ctrl Pts',(21.4872825238012,19.9608442409695,-16.4481274320642));
#120355=CARTESIAN_POINT('Ctrl Pts',(20.854799951232,17.3018015796049,-16.5753032387457));
#120356=CARTESIAN_POINT('Ctrl Pts',(18.2766150550976,16.3943299707347,-16.7024790454271));
#120357=CARTESIAN_POINT('Ctrl Pts',(16.1180524573998,18.0709782914572,-16.8296548521085));
#120358=CARTESIAN_POINT('Ctrl Pts',(16.3594593660219,20.7935257720403,-16.9568306587899));
#120359=CARTESIAN_POINT('Ctrl Pts',(18.7793599257057,22.0642040794035,-17.0840064654714));
#120360=CARTESIAN_POINT('Ctrl Pts',(21.1576455689089,20.717244733731,-17.2111822721528));
#120361=CARTESIAN_POINT('Ctrl Pts',(21.3123868310473,17.9883993329521,-17.3383580788343));
#120362=CARTESIAN_POINT('Ctrl Pts',(19.1016182084348,16.3812141610339,-17.4655338855157));
#120363=CARTESIAN_POINT('Ctrl Pts',(16.5535826965425,17.3701818600505,-17.5927096921971));
#120364=CARTESIAN_POINT('Ctrl Pts',(16.0059447286121,20.0479859484101,-17.7198854988786));
#120365=CARTESIAN_POINT('Ctrl Pts',(17.9611281499736,21.9579073783129,-17.84706130556));
#120366=CARTESIAN_POINT('Ctrl Pts',(20.6253735238976,21.3477117809083,-17.9742371122414));
#120367=CARTESIAN_POINT('Ctrl Pts',(21.5544010815252,18.7772157438201,-18.1014129189229));
#120368=CARTESIAN_POINT('Ctrl Pts',(19.8958857006878,16.6046898380703,-18.2285887256043));
#120369=CARTESIAN_POINT('Ctrl Pts',(17.1714123042272,16.8232917400757,-18.3557645322858));
#120370=CARTESIAN_POINT('Ctrl Pts',(15.8805161335109,19.2324677726021,-18.4829403389672));
#120371=CARTESIAN_POINT('Ctrl Pts',(17.2075143031097,21.6219484563437,-18.6101161456486));
#120372=CARTESIAN_POINT('Ctrl Pts',(19.9349683552291,21.7995335714625,-18.7372919523301));
#120373=CARTESIAN_POINT('Ctrl Pts',(21.5606084819066,19.6022997977881,-18.8644677590115));
#120374=CARTESIAN_POINT('Ctrl Pts',(20.5930107655851,17.0460727454631,-18.9916435656929));
#120375=CARTESIAN_POINT('Ctrl Pts',(17.919886054979,16.4760320805331,-19.1188193723744));
#120376=CARTESIAN_POINT('Ctrl Pts',(15.9936603594759,18.4151547268051,-19.2459951790558));
#120377=CARTESIAN_POINT('Ctrl Pts',(16.5815261991922,21.0844160225493,-19.3731709857372));
#120378=CARTESIAN_POINT('Ctrl Pts',(19.1441531541393,22.0349343813413,-19.5003467924186));
#120379=CARTESIAN_POINT('Ctrl Pts',(21.3304900460201,20.3946682445481,-19.6275225991001));
#120380=CARTESIAN_POINT('Ctrl Pts',(21.1347084791815,17.6684599097052,-19.7546984057815));
#120381=CARTESIAN_POINT('Ctrl Pts',(18.7364258833105,16.3574364640233,-19.8818742124629));
#120382=CARTESIAN_POINT('Ctrl Pts',(16.3359176980786,17.6643802632539,-20.0090500191444));
#120383=CARTESIAN_POINT('Ctrl Pts',(16.1355011676512,20.3902520376885,-20.1362258258258));
#120384=CARTESIAN_POINT('Ctrl Pts',(18.3190460646205,22.0342325649128,-20.2634016325072));
#120385=CARTESIAN_POINT('Ctrl Pts',(20.8832853850366,21.0880737832455,-20.3905774391887));
#120386=CARTESIAN_POINT('Ctrl Pts',(21.4756888748341,18.4198137277981,-20.5177532458701));
#120387=CARTESIAN_POINT('Ctrl Pts',(19.5527627775141,16.4774229462598,-20.6449290525516));
#120388=CARTESIAN_POINT('Ctrl Pts',(16.8786730601742,17.0429098579489,-20.772104859233));
#120389=CARTESIAN_POINT('Ctrl Pts',(15.9067298650559,19.5975033862937,-20.8992806659144));
#120390=CARTESIAN_POINT('Ctrl Pts',(17.5286330619216,21.7974684377538,-21.0264564725959));
#120391=CARTESIAN_POINT('Ctrl Pts',(20.2563826753269,21.6245778537434,-21.1536322792773));
#120392=CARTESIAN_POINT('Ctrl Pts',(21.5874463311991,19.2372471517761,-21.2808080859587));
#120393=CARTESIAN_POINT('Ctrl Pts',(20.300639179667,16.8260911603011,-21.4079838926401));
#120394=CARTESIAN_POINT('Ctrl Pts',(17.5765588401915,16.6024498642088,-21.5351596993216));
#120395=CARTESIAN_POINT('Ctrl Pts',(15.9143183086354,18.7729382233993,-21.662335506003));
#120396=CARTESIAN_POINT('Ctrl Pts',(16.8390399827,21.3434932755793,-21.7895113126845));
#120397=CARTESIAN_POINT('Ctrl Pts',(19.5021077373455,21.9611708420245,-21.9166871193659));
#120398=CARTESIAN_POINT('Ctrl Pts',(21.4611725520066,20.0483226159722,-22.0438815838219));
#120399=CARTESIAN_POINT('Ctrl Pts',(21.097729963592,18.2714051422367,-22.1286841127175));
#120400=CARTESIAN_POINT('Ctrl Pts',(20.5799309194189,17.6565535467265,-22.1710947060526));
#120401=CARTESIAN_POINT('Ctrl Pts',(18.1489776472236,17.0246983287242,0.17134583652952));
#120402=CARTESIAN_POINT('Ctrl Pts',(17.4210583805961,17.2194788787227,0.128953900969042));
#120403=CARTESIAN_POINT('Ctrl Pts',(16.1877700772709,18.3901108027545,0.0441700298480857));
#120404=CARTESIAN_POINT('Ctrl Pts',(16.6662106099602,20.9125930681132,-0.0830057768333481));
#120405=CARTESIAN_POINT('Ctrl Pts',(19.0452436430351,21.8682695891329,-0.210181583514783));
#120406=CARTESIAN_POINT('Ctrl Pts',(21.1369461627689,20.3888844472776,-0.337357390196217));
#120407=CARTESIAN_POINT('Ctrl Pts',(21.0250156242086,17.8274157338044,-0.464533196877652));
#120408=CARTESIAN_POINT('Ctrl Pts',(18.8107430744499,16.5360493895473,-0.591709003559086));
#120409=CARTESIAN_POINT('Ctrl Pts',(16.5263111813342,17.6983953463737,-0.71888481024052));
#120410=CARTESIAN_POINT('Ctrl Pts',(16.2671682429258,20.2486639579588,-0.846060616921954));
#120411=CARTESIAN_POINT('Ctrl Pts',(18.271257019252,21.8468355936962,-0.97323642360339));
#120412=CARTESIAN_POINT('Ctrl Pts',(20.6998491546166,21.0268460006587,-1.10041223028482));
#120413=CARTESIAN_POINT('Ctrl Pts',(21.3249146619818,18.5409022133311,-1.22758803696626));
#120414=CARTESIAN_POINT('Ctrl Pts',(19.5729674590718,16.669746184055,-1.35476384364769));
#120415=CARTESIAN_POINT('Ctrl Pts',(17.0513245200395,17.1300252112755,-1.48193965032912));
#120416=CARTESIAN_POINT('Ctrl Pts',(16.0734293860861,19.4994733867219,-1.60911545701056));
#120417=CARTESIAN_POINT('Ctrl Pts',(17.5364439588135,21.6042630902867,-1.73629126369199));
#120418=CARTESIAN_POINT('Ctrl Pts',(20.0981411949616,21.5133835119668,-1.86346707037343));
#120419=CARTESIAN_POINT('Ctrl Pts',(21.4083239034943,19.3102094129899,-1.99064287705486));
#120420=CARTESIAN_POINT('Ctrl Pts',(20.2649802358942,17.0160171208712,-2.1178186837363));
#120421=CARTESIAN_POINT('Ctrl Pts',(17.7170573196222,16.7355852361245,-2.24499449041773));
#120422=CARTESIAN_POINT('Ctrl Pts',(16.1021161450239,18.7261928325832,-2.37217029709916));
#120423=CARTESIAN_POINT('Ctrl Pts',(16.9017650796541,21.1615808747066,-2.4993461037806));
#120424=CARTESIAN_POINT('Ctrl Pts',(19.3823758191848,21.8074320517016,-2.62652191046204));
#120425=CARTESIAN_POINT('Ctrl Pts',(21.2681419942009,20.0712179632603,-2.75369771714347));
#120426=CARTESIAN_POINT('Ctrl Pts',(20.8289901725761,17.5458072902532,-2.8808735238249));
#120427=CARTESIAN_POINT('Ctrl Pts',(18.4678148992109,16.5481075720289,-3.00804933050634));
#120428=CARTESIAN_POINT('Ctrl Pts',(16.3508479335524,17.9934463802261,-3.13522513718777));
#120429=CARTESIAN_POINT('Ctrl Pts',(16.420275074257,20.5558150638861,-3.26240094386921));
#120430=CARTESIAN_POINT('Ctrl Pts',(18.6124012281085,21.8843993954715,-3.38957675055063));
#120431=CARTESIAN_POINT('Ctrl Pts',(20.9160867080332,20.7603057113818,-3.51675255723208));
#120432=CARTESIAN_POINT('Ctrl Pts',(21.2178430688434,18.2148201979656,-3.64392836391351));
#120433=CARTESIAN_POINT('Ctrl Pts',(19.2408275787131,16.5832678229678,-3.77110417059494));
#120434=CARTESIAN_POINT('Ctrl Pts',(16.7988292423621,17.3624966249737,-3.89827997727638));
#120435=CARTESIAN_POINT('Ctrl Pts',(16.1322299659104,19.8376125424924,-4.02545578395781));
#120436=CARTESIAN_POINT('Ctrl Pts',(17.8525932116705,21.7378503442427,-4.15263159063924));
#120437=CARTESIAN_POINT('Ctrl Pts',(20.3815924794505,21.3198597891662,-4.27980739732068));
#120438=CARTESIAN_POINT('Ctrl Pts',(21.3990279084555,18.9671212681321,-4.40698320400211));
#120439=CARTESIAN_POINT('Ctrl Pts',(19.97146564174,16.8381263467644,-4.53415901068355));
#120440=CARTESIAN_POINT('Ctrl Pts',(17.4086054545075,16.8860957250923,-4.66133481736498));
#120441=CARTESIAN_POINT('Ctrl Pts',(16.0617124995014,19.0670204758143,-4.78851062404641));
#120442=CARTESIAN_POINT('Ctrl Pts',(17.1664774653348,21.3800375035998,-4.91568643072785));
#120443=CARTESIAN_POINT('Ctrl Pts',(19.7093470653026,21.7030972474828,-5.04286223740928));
#120444=CARTESIAN_POINT('Ctrl Pts',(21.3573962697213,19.7398124437998,-5.17003804409073));
#120445=CARTESIAN_POINT('Ctrl Pts',(20.5986422230066,17.2913750447324,-5.29721385077215));
#120446=CARTESIAN_POINT('Ctrl Pts',(18.1291946694319,16.6040743967613,-5.42438965745359));
#120447=CARTESIAN_POINT('Ctrl Pts',(16.214618468201,18.3084661857105,-5.55156546413503));
#120448=CARTESIAN_POINT('Ctrl Pts',(16.6114184519424,20.8408767317044,-5.67874127081646));
#120449=CARTESIAN_POINT('Ctrl Pts',(18.9555552637581,21.8779765379183,-5.80591707749789));
#120450=CARTESIAN_POINT('Ctrl Pts',(21.0964288723461,20.4682909018246,-5.93309288417933));
#120451=CARTESIAN_POINT('Ctrl Pts',(21.069920619429,17.905118899581,-6.06026869086075));
#120452=CARTESIAN_POINT('Ctrl Pts',(18.9003501817706,16.5400117548499,-6.1874444975422));
#120453=CARTESIAN_POINT('Ctrl Pts',(16.5781637771942,17.6253705448169,-6.31462030422363));
#120454=CARTESIAN_POINT('Ctrl Pts',(16.2338233007557,20.1654459446513,-6.44179611090507));
#120455=CARTESIAN_POINT('Ctrl Pts',(18.1832397674068,21.8298764298645,-6.5689719175865));
#120456=CARTESIAN_POINT('Ctrl Pts',(20.637944563427,21.09165033648,-6.69614772426794));
#120457=CARTESIAN_POINT('Ctrl Pts',(21.3458983946297,18.6280442856993,-6.82332353094937));
#120458=CARTESIAN_POINT('Ctrl Pts',(19.657597561457,16.6992639204773,-6.9504993376308));
#120459=CARTESIAN_POINT('Ctrl Pts',(17.1219532905771,17.0748455122945,-7.07767514431223));
#120460=CARTESIAN_POINT('Ctrl Pts',(16.0652618206899,19.4102162618813,-7.20485095099367));
#120461=CARTESIAN_POINT('Ctrl Pts',(17.4569719897474,21.5628184559476,-7.3320267576751));
#120462=CARTESIAN_POINT('Ctrl Pts',(20.0202760969144,21.5577731869978,-7.45920256435654));
#120463=CARTESIAN_POINT('Ctrl Pts',(21.4035017204607,19.3997091761485,-7.58637837103798));
#120464=CARTESIAN_POINT('Ctrl Pts',(20.3376252034471,17.0685162087954,-7.7135541777194));
#120465=CARTESIAN_POINT('Ctrl Pts',(17.8005220944761,16.7029191423313,-7.84072998440084));
#120466=CARTESIAN_POINT('Ctrl Pts',(16.1198270256501,18.638330593724,-7.96790579108227));
#120467=CARTESIAN_POINT('Ctrl Pts',(16.8374734069165,21.099130681503,-8.09508159776372));
#120468=CARTESIAN_POINT('Ctrl Pts',(19.2950652256212,21.8276880596097,-8.22225740444514));
#120469=CARTESIAN_POINT('Ctrl Pts',(21.2379145234536,20.155596553002,-8.34943321112658));
#120470=CARTESIAN_POINT('Ctrl Pts',(20.8835776564797,17.616896337289,-8.47660901780802));
#120471=CARTESIAN_POINT('Ctrl Pts',(18.5571367075217,16.5406872908817,-8.60378482448944));
#120472=CARTESIAN_POINT('Ctrl Pts',(16.3929568520385,17.9143244167918,-8.73096063117089));
#120473=CARTESIAN_POINT('Ctrl Pts',(16.3765387832853,20.4775809095322,-8.85813643785231));
#120474=CARTESIAN_POINT('Ctrl Pts',(18.5229450603227,21.878828030654,-8.98531224453375));
#120475=CARTESIAN_POINT('Ctrl Pts',(20.8629811449671,20.8325085177327,-9.11248805121519));
#120476=CARTESIAN_POINT('Ctrl Pts',(21.2498091685766,18.2985555819606,-9.23966385789662));
#120477=CARTESIAN_POINT('Ctrl Pts',(19.3285384287442,16.6017137670521,-9.36683966457805));
#120478=CARTESIAN_POINT('Ctrl Pts',(16.8618155817557,17.2987301203051,-9.49401547125949));
#120479=CARTESIAN_POINT('Ctrl Pts',(16.1127057376362,19.7501353993238,-9.62119127794092));
#120480=CARTESIAN_POINT('Ctrl Pts',(17.7684706833649,21.7069174119797,-9.74836708462235));
#120481=CARTESIAN_POINT('Ctrl Pts',(20.3100488495983,21.3738501132499,-9.87554289130379));
#120482=CARTESIAN_POINT('Ctrl Pts',(21.405700016949,19.0565020772309,-10.0027186979853));
#120483=CARTESIAN_POINT('Ctrl Pts',(20.0502322431535,16.8808962961301,-10.1298945046666));
#120484=CARTESIAN_POINT('Ctrl Pts',(17.487203080851,16.8430160407836,-10.2570703113481));
#120485=CARTESIAN_POINT('Ctrl Pts',(16.0680327069235,18.9776140943582,-10.3842461180296));
#120486=CARTESIAN_POINT('Ctrl Pts',(17.0947218558021,21.3263292307962,-10.511421924711));
#120487=CARTESIAN_POINT('Ctrl Pts',(19.6253469569058,21.7343610901177,-10.6385977313924));
#120488=CARTESIAN_POINT('Ctrl Pts',(21.3382165482799,19.8273657667087,-10.7657735380739));
#120489=CARTESIAN_POINT('Ctrl Pts',(20.6618790925152,17.3548931083184,-10.8929493447553));
#120490=CARTESIAN_POINT('Ctrl Pts',(18.2168322270393,16.5852833200598,-11.0201251514367));
#120491=CARTESIAN_POINT('Ctrl Pts',(16.2462546942025,18.2246056152896,-11.1473009581181));
#120492=CARTESIAN_POINT('Ctrl Pts',(16.5580290725475,20.768883535951,-11.2744767647995));
#120493=CARTESIAN_POINT('Ctrl Pts',(18.8661217208428,21.8839000055346,-11.401652571481));
#120494=CARTESIAN_POINT('Ctrl Pts',(21.0530008906637,20.5466966189245,-11.5288283781625));
#120495=CARTESIAN_POINT('Ctrl Pts',(21.1123406767285,17.984074487133,-11.6560041848439));
#120496=CARTESIAN_POINT('Ctrl Pts',(18.9897005083654,16.5470803618114,-11.7831799915254));
#120497=CARTESIAN_POINT('Ctrl Pts',(16.6324709941403,17.554067163028,-11.9103557982068));
#120498=CARTESIAN_POINT('Ctrl Pts',(16.2032639071911,20.0811870013163,-12.0375316048882));
#120499=CARTESIAN_POINT('Ctrl Pts',(18.0958501101972,21.8099642757934,-12.1647074115696));
#120500=CARTESIAN_POINT('Ctrl Pts',(20.5738992290484,21.1543531371454,-12.291883218251));
#120501=CARTESIAN_POINT('Ctrl Pts',(21.3639550022726,18.7158361132654,-12.4190590249325));
#120502=CARTESIAN_POINT('Ctrl Pts',(19.7411902943285,16.7316012221275,-12.546234831614));
#120503=CARTESIAN_POINT('Ctrl Pts',(17.1943910046178,17.0220608208441,-12.6734106382954));
#120504=CARTESIAN_POINT('Ctrl Pts',(16.0600874092589,19.3207362555485,-12.8005864449768));
#120505=CARTESIAN_POINT('Ctrl Pts',(17.3789326541725,21.5187354867873,-12.9277622516583));
#120506=CARTESIAN_POINT('Ctrl Pts',(19.940968083918,21.5995306431169,-13.0549380583397));
#120507=CARTESIAN_POINT('Ctrl Pts',(21.3956852095567,19.4889971833178,-13.1821138650211));
#120508=CARTESIAN_POINT('Ctrl Pts',(20.4084713582425,17.1234185622757,-13.3092896717026));
#120509=CARTESIAN_POINT('Ctrl Pts',(17.8850339651544,16.6730663404289,-13.436465478384));
#120510=CARTESIAN_POINT('Ctrl Pts',(16.1404702162623,18.5511107293104,-13.5636412850654));
#120511=CARTESIAN_POINT('Ctrl Pts',(16.7753090713368,21.0345625667023,-13.6908170917469));
#120512=CARTESIAN_POINT('Ctrl Pts',(19.2071252833902,21.8450089322025,-13.8179928984283));
#120513=CARTESIAN_POINT('Ctrl Pts',(21.2048784133999,20.2389155874388,-13.9451687051096));
#120514=CARTESIAN_POINT('Ctrl Pts',(20.9357539591253,17.6897734908367,-14.0723445117912));
#120515=CARTESIAN_POINT('Ctrl Pts',(18.6466569036158,16.5362622984264,-14.1995203184726));
#120516=CARTESIAN_POINT('Ctrl Pts',(16.4376917179148,17.8366569342653,-14.326696125154));
#120517=CARTESIAN_POINT('Ctrl Pts',(16.3354468560612,20.3979260315651,-14.4538719318355));
#120518=CARTESIAN_POINT('Ctrl Pts',(18.4337256327737,21.8702641638416,-14.5810477385169));
#120519=CARTESIAN_POINT('Ctrl Pts',(20.8074875042872,20.9028924783419,-14.7082235451983));
#120520=CARTESIAN_POINT('Ctrl Pts',(21.2789532857658,18.3833144546537,-14.8353993518798));
#120521=CARTESIAN_POINT('Ctrl Pts',(19.4155823851695,16.6230865468621,-14.9625751585612));
#120522=CARTESIAN_POINT('Ctrl Pts',(16.9269019499539,17.2371086083006,-15.0897509652427));
#120523=CARTESIAN_POINT('Ctrl Pts',(16.0961218145012,19.6620535081066,-15.2169267719241));
#120524=CARTESIAN_POINT('Ctrl Pts',(17.6854311890587,21.6731848097627,-15.3441025786055));
#120525=CARTESIAN_POINT('Ctrl Pts',(20.2367373661345,21.425414368886,-15.4712783852869));
#120526=CARTESIAN_POINT('Ctrl Pts',(21.4093752801818,19.1460561866125,-15.5984541919684));
#120527=CARTESIAN_POINT('Ctrl Pts',(20.1275224271794,16.9262799222545,-15.7256299986498));
#120528=CARTESIAN_POINT('Ctrl Pts',(17.5671992389961,16.8025925235073,-15.8528058053313));
#120529=CARTESIAN_POINT('Ctrl Pts',(16.0773433292112,18.8884695018156,-15.9799816120127));
#120530=CARTESIAN_POINT('Ctrl Pts',(17.0248050241658,21.2702481937078,-16.1071574186941));
#120531=CARTESIAN_POINT('Ctrl Pts',(19.5403470248439,21.7627944792304,-16.2343332253756));
#120532=CARTESIAN_POINT('Ctrl Pts',(21.3161156777683,19.9142277122867,-16.361509032057));
#120533=CARTESIAN_POINT('Ctrl Pts',(20.7229534605137,17.4204931665544,-16.4886848387384));
#120534=CARTESIAN_POINT('Ctrl Pts',(18.3050498916118,16.5694375091209,-16.6158606454198));
#120535=CARTESIAN_POINT('Ctrl Pts',(16.2806814235098,18.1418514832104,-16.7430364521013));
#120536=CARTESIAN_POINT('Ctrl Pts',(16.5070804792137,20.6951428626135,-16.8702122587827));
#120537=CARTESIAN_POINT('Ctrl Pts',(18.7765399770255,21.8868252818636,-16.9973880654642));
#120538=CARTESIAN_POINT('Ctrl Pts',(21.0069716862451,20.6236040854512,-17.1245638721456));
#120539=CARTESIAN_POINT('Ctrl Pts',(21.1520929498682,18.0644063167351,-17.251739678827));
#120540=CARTESIAN_POINT('Ctrl Pts',(19.0787640157619,16.5571370867842,-17.3789154855085));
#120541=CARTESIAN_POINT('Ctrl Pts',(16.6891354956622,17.4846223624005,-17.5060912921899));
#120542=CARTESIAN_POINT('Ctrl Pts',(16.1755432396875,19.9959519694325,-17.6332670988714));
#120543=CARTESIAN_POINT('Ctrl Pts',(18.0091762655641,21.7871368641264,-17.7604429055528));
#120544=CARTESIAN_POINT('Ctrl Pts',(20.5077900801511,21.2148760790659,-17.8876187122342));
#120545=CARTESIAN_POINT('Ctrl Pts',(21.3790615900277,18.8041833660481,-18.0147945189156));
#120546=CARTESIAN_POINT('Ctrl Pts',(19.8236532620919,16.7667196647752,-18.1419703255971));
#120547=CARTESIAN_POINT('Ctrl Pts',(17.2685556976942,16.9717314619586,-18.2691461322785));
#120548=CARTESIAN_POINT('Ctrl Pts',(16.0579123249335,19.231133158048,-18.3963219389599));
#120549=CARTESIAN_POINT('Ctrl Pts',(17.3024132973075,21.4720639313621,-18.5234977456414));
#120550=CARTESIAN_POINT('Ctrl Pts',(19.8603062151207,21.6386088848577,-18.6506735523228));
#120551=CARTESIAN_POINT('Ctrl Pts',(21.3848830869879,19.5779733613755,-18.7778493590042));
#120552=CARTESIAN_POINT('Ctrl Pts',(20.4774392589433,17.1806625548439,-18.9050251656857));
#120553=CARTESIAN_POINT('Ctrl Pts',(17.9704981207863,16.6460603390679,-19.0322009723671));
#120554=CARTESIAN_POINT('Ctrl Pts',(16.1640225686834,18.4646310606594,-19.1593767790485));
#120555=CARTESIAN_POINT('Ctrl Pts',(16.7153417987421,20.9679489658214,-19.28655258573));
#120556=CARTESIAN_POINT('Ctrl Pts',(19.1186546369411,21.8593752306623,-19.4137283924114));
#120557=CARTESIAN_POINT('Ctrl Pts',(21.1690707190565,20.3210816226097,-19.5409041990928));
#120558=CARTESIAN_POINT('Ctrl Pts',(20.985460555994,17.7643569779692,-19.6680800057743));
#120559=CARTESIAN_POINT('Ctrl Pts',(18.7362750703113,16.5348376083611,-19.7952558124557));
#120560=CARTESIAN_POINT('Ctrl Pts',(16.485002356336,17.7605309561315,-19.9224316191372));
#120561=CARTESIAN_POINT('Ctrl Pts',(16.2970453774111,20.3169399637462,-20.0496074258186));
#120562=CARTESIAN_POINT('Ctrl Pts',(18.3448430381436,21.8587170449558,-20.1767832325));
#120563=CARTESIAN_POINT('Ctrl Pts',(20.7496680038194,20.9713793298171,-20.3039590391814));
#120564=CARTESIAN_POINT('Ctrl Pts',(21.3052427860467,18.4690004195621,-20.4311348458629));
#120565=CARTESIAN_POINT('Ctrl Pts',(19.5018617017747,16.6473647370611,-20.5583106525443));
#120566=CARTESIAN_POINT('Ctrl Pts',(16.9940155496951,17.1776962986144,-20.6854864592258));
#120567=CARTESIAN_POINT('Ctrl Pts',(16.0824963938076,19.5734751345466,-20.8126622659072));
#120568=CARTESIAN_POINT('Ctrl Pts',(17.6035686543715,21.6366721369649,-20.9398380725886));
#120569=CARTESIAN_POINT('Ctrl Pts',(20.1617387589333,21.4745298636412,-21.0670138792701));
#120570=CARTESIAN_POINT('Ctrl Pts',(21.4100524732811,19.2356154114268,-21.1941896859515));
#120571=CARTESIAN_POINT('Ctrl Pts',(20.2032439124044,16.9743568470362,-21.3213654926329));
#120572=CARTESIAN_POINT('Ctrl Pts',(17.6485149693138,16.7646189462416,-21.4485412993143));
#120573=CARTESIAN_POINT('Ctrl Pts',(16.0896130768821,18.8001717717257,-21.5757171059958));
#120574=CARTESIAN_POINT('Ctrl Pts',(16.9568463925819,21.2109198309685,-21.7028929126772));
#120575=CARTESIAN_POINT('Ctrl Pts',(19.4543557984586,21.7901974439036,-21.8300687193587));
#120576=CARTESIAN_POINT('Ctrl Pts',(21.2916289180791,19.9962677069502,-21.9572631838147));
#120577=CARTESIAN_POINT('Ctrl Pts',(20.950780931212,18.329818140889,-22.0420657127103));
#120578=CARTESIAN_POINT('Ctrl Pts',(20.46517256435,17.753190813129,-22.0844763060453));
#120579=CARTESIAN_POINT('Ctrl Pts',(18.1877584159729,17.169626909876,0.257964236536772));
#120580=CARTESIAN_POINT('Ctrl Pts',(17.5080924658439,17.3514955780797,0.215572300976294));
#120581=CARTESIAN_POINT('Ctrl Pts',(16.3565580788699,18.4445270382643,0.130788429855338));
#120582=CARTESIAN_POINT('Ctrl Pts',(16.8032830855277,20.7997955194952,0.00361262317390322));
#120583=CARTESIAN_POINT('Ctrl Pts',(19.0246114950703,21.6921208369499,-0.123563183507531));
#120584=CARTESIAN_POINT('Ctrl Pts',(20.9776563527076,20.3108032181647,-0.250738990188965));
#120585=CARTESIAN_POINT('Ctrl Pts',(20.8731456200936,17.9191326762732,-0.3779147968704));
#120586=CARTESIAN_POINT('Ctrl Pts',(18.8056558236651,16.7133702056622,-0.505090603551834));
#120587=CARTESIAN_POINT('Ctrl Pts',(16.6726575032154,17.7986649702659,-0.632266410233268));
#120588=CARTESIAN_POINT('Ctrl Pts',(16.4306929893915,20.1798778580737,-0.759442216914702));
#120589=CARTESIAN_POINT('Ctrl Pts',(18.301931964306,21.6721076877706,-0.886618023596137));
#120590=CARTESIAN_POINT('Ctrl Pts',(20.5695342339997,20.9064746960381,-1.01379383027757));
#120591=CARTESIAN_POINT('Ctrl Pts',(21.1531645367453,18.5853225798024,-1.140969636959));
#120592=CARTESIAN_POINT('Ctrl Pts',(19.5173528268034,16.8382043226231,-1.26814544364043));
#120593=CARTESIAN_POINT('Ctrl Pts',(17.1628680334775,17.2679717387401,-1.39532125032187));
#120594=CARTESIAN_POINT('Ctrl Pts',(16.2497969611534,19.4803506649187,-1.5224970570033));
#120595=CARTESIAN_POINT('Ctrl Pts',(17.6158292056801,21.4456151650917,-1.64967286368474));
#120596=CARTESIAN_POINT('Ctrl Pts',(20.0077131216202,21.3607599376264,-1.77684867036617));
#120597=CARTESIAN_POINT('Ctrl Pts',(21.2310446313948,19.3036328825639,-1.90402447704761));
#120598=CARTESIAN_POINT('Ctrl Pts',(20.1634925060559,17.1615211739047,-2.03120028372904));
#120599=CARTESIAN_POINT('Ctrl Pts',(17.7844698188743,16.8996789447851,-2.15837609041048));
#120600=CARTESIAN_POINT('Ctrl Pts',(16.2765820926419,18.7583303988802,-2.28555189709191));
#120601=CARTESIAN_POINT('Ctrl Pts',(17.0232227955911,21.0322780788906,-2.41272770377335));
#120602=CARTESIAN_POINT('Ctrl Pts',(19.3393953884592,21.6353161821242,-2.53990351045478));
#120603=CARTESIAN_POINT('Ctrl Pts',(21.1001552938832,20.0141946482555,-2.66707931713621));
#120604=CARTESIAN_POINT('Ctrl Pts',(20.6901145740129,17.6561918817021,-2.79425512381765));
#120605=CARTESIAN_POINT('Ctrl Pts',(18.4854601443698,16.7246290587094,-2.92143093049908));
#120606=CARTESIAN_POINT('Ctrl Pts',(16.5088256052511,18.0741572541683,-3.04860673718052));
#120607=CARTESIAN_POINT('Ctrl Pts',(16.5736504638791,20.4666681077815,-3.17578254386197));
#120608=CARTESIAN_POINT('Ctrl Pts',(18.6204619352431,21.7071814084352,-3.30295835054339));
#120609=CARTESIAN_POINT('Ctrl Pts',(20.7714375341794,20.6576031971447,-3.43013415722482));
#120610=CARTESIAN_POINT('Ctrl Pts',(21.0531906530764,18.2808563388961,-3.55730996390625));
#120611=CARTESIAN_POINT('Ctrl Pts',(19.2072302930153,16.7574585584311,-3.6844857705877));
#120612=CARTESIAN_POINT('Ctrl Pts',(16.9271105110797,17.4850327666767,-3.81166157726912));
#120613=CARTESIAN_POINT('Ctrl Pts',(16.3046996870279,19.7960747858742,-3.93883738395056));
#120614=CARTESIAN_POINT('Ctrl Pts',(17.911021120741,21.5703470028761,-4.066013190632));
#120615=CARTESIAN_POINT('Ctrl Pts',(20.2723745963467,21.1800647823256,-4.19318899731344));
#120616=CARTESIAN_POINT('Ctrl Pts',(21.2223648620988,18.9832878379367,-4.32036480399487));
#120617=CARTESIAN_POINT('Ctrl Pts',(19.8894348122174,16.9954226688293,-4.44754061067631));
#120618=CARTESIAN_POINT('Ctrl Pts',(17.4964650364985,17.0402121868336,-4.57471641735773));
#120619=CARTESIAN_POINT('Ctrl Pts',(16.23885677971,19.0765647891309,-4.70189222403917));
#120620=CARTESIAN_POINT('Ctrl Pts',(17.2703875614835,21.2362533534106,-4.8290680307206));
#120621=CARTESIAN_POINT('Ctrl Pts',(19.6446919135629,21.5378976673356,-4.95624383740204));
#120622=CARTESIAN_POINT('Ctrl Pts',(21.1834929588632,19.7047577950374,-5.08341964408348));
#120623=CARTESIAN_POINT('Ctrl Pts',(20.4750362470855,17.4186257918574,-5.21059545076491));
#120624=CARTESIAN_POINT('Ctrl Pts',(18.1692868395033,16.7768858773585,-5.33777125744635));
#120625=CARTESIAN_POINT('Ctrl Pts',(16.3816267066251,18.3682945922223,-5.46494706412778));
#120626=CARTESIAN_POINT('Ctrl Pts',(16.7521230656655,20.7328332145257,-5.59212287080921));
#120627=CARTESIAN_POINT('Ctrl Pts',(18.9408685028023,21.7011843181237,-5.71929867749065));
#120628=CARTESIAN_POINT('Ctrl Pts',(20.9398249283253,20.3849458681128,-5.84647448417208));
#120629=CARTESIAN_POINT('Ctrl Pts',(20.9150738910453,17.9916849474066,-5.97365029085351));
#120630=CARTESIAN_POINT('Ctrl Pts',(18.889322931444,16.7170699082275,-6.10082609753496));
#120631=CARTESIAN_POINT('Ctrl Pts',(16.7210728226713,17.7304809374911,-6.22800190421637));
#120632=CARTESIAN_POINT('Ctrl Pts',(16.3995584627467,20.1021763152302,-6.35517771089783));
#120633=CARTESIAN_POINT('Ctrl Pts',(18.2197493214694,21.6562727363857,-6.48235351757925));
#120634=CARTESIAN_POINT('Ctrl Pts',(20.5117332597471,20.96698319265,-6.6095293242607));
#120635=CARTESIAN_POINT('Ctrl Pts',(21.1727572707768,18.6666880582664,-6.73670513094212));
#120636=CARTESIAN_POINT('Ctrl Pts',(19.5963728522159,16.8657653466142,-6.86388093762356));
#120637=CARTESIAN_POINT('Ctrl Pts',(17.2288148666425,17.2164498677646,-6.99105674430498));
#120638=CARTESIAN_POINT('Ctrl Pts',(16.2421708185993,19.3970103394982,-7.11823255098643));
#120639=CARTESIAN_POINT('Ctrl Pts',(17.5416253841297,21.406917869846,-7.24540835766785));
#120640=CARTESIAN_POINT('Ctrl Pts',(19.935009652606,21.4022070486441,-7.3725841643493));
#120641=CARTESIAN_POINT('Ctrl Pts',(21.2265421078823,19.3871997619589,-7.49975997103072));
#120642=CARTESIAN_POINT('Ctrl Pts',(20.2313218837872,17.210540129867,-7.62693577771217));
#120643=CARTESIAN_POINT('Ctrl Pts',(17.8624017655944,16.8691782660797,-7.75411158439359));
#120644=CARTESIAN_POINT('Ctrl Pts',(16.2931189299813,18.676292493315,-7.88128739107503));
#120645=CARTESIAN_POINT('Ctrl Pts',(16.9631929779452,20.9739676702432,-8.00846319775646));
#120646=CARTESIAN_POINT('Ctrl Pts',(19.2578725599652,21.6542294318373,-8.13563900443789));
#120647=CARTESIAN_POINT('Ctrl Pts',(21.0719315834152,20.0929798336416,-8.26281481111933));
#120648=CARTESIAN_POINT('Ctrl Pts',(20.7410834874809,17.7225684799219,-8.38999061780077));
#120649=CARTESIAN_POINT('Ctrl Pts',(18.5688608654335,16.7177006633949,-8.5171664244822));
#120650=CARTESIAN_POINT('Ctrl Pts',(16.5481431496601,18.0002802365935,-8.64434223116363));
#120651=CARTESIAN_POINT('Ctrl Pts',(16.5328134244968,20.3936200469742,-8.77151803784506));
#120652=CARTESIAN_POINT('Ctrl Pts',(18.5369357613108,21.7019793659344,-8.89869384452652));
#120653=CARTESIAN_POINT('Ctrl Pts',(20.721852305936,20.7250197242656,-9.02586965120793));
#120654=CARTESIAN_POINT('Ctrl Pts',(21.0830377398936,18.3590409562453,-9.15304545788938));
#120655=CARTESIAN_POINT('Ctrl Pts',(19.2891268452239,16.774681732328,-9.2802212645708));
#120656=CARTESIAN_POINT('Ctrl Pts',(16.985921525119,17.4254933040343,-9.40739707125225));
#120657=CARTESIAN_POINT('Ctrl Pts',(16.2864697077309,19.7143964482452,-9.53457287793367));
#120658=CARTESIAN_POINT('Ctrl Pts',(17.8324750226373,21.5414645954985,-9.66174868461511));
#120659=CARTESIAN_POINT('Ctrl Pts',(20.2055735493235,21.2304761213276,-9.78892449129655));
#120660=CARTESIAN_POINT('Ctrl Pts',(21.2285946806605,19.0667436486627,-9.91610029797797));
#120661=CARTESIAN_POINT('Ctrl Pts',(19.9629800244992,17.0353574247909,-10.0432761046594));
#120662=CARTESIAN_POINT('Ctrl Pts',(17.5698524749629,16.999988228066,-10.1704519113408));
#120663=CARTESIAN_POINT('Ctrl Pts',(16.2447580245038,18.9930851012233,-10.2976277180222));
#120664=CARTESIAN_POINT('Ctrl Pts',(17.2033885867812,21.1861053686842,-10.4248035247037));
#120665=CARTESIAN_POINT('Ctrl Pts',(19.5662601202284,21.567089049242,-10.5519793313851));
#120666=CARTESIAN_POINT('Ctrl Pts',(21.1655846492548,19.786507262499,-10.6791551380666));
#120667=CARTESIAN_POINT('Ctrl Pts',(20.534081183754,17.4779332824223,-10.806330944748));
#120668=CARTESIAN_POINT('Ctrl Pts',(18.2511149577974,16.7593404494715,-10.9335067514294));
#120669=CARTESIAN_POINT('Ctrl Pts',(16.4111657868359,18.2899930869776,-11.0606825581108));
#120670=CARTESIAN_POINT('Ctrl Pts',(16.7022728351016,20.6656124030459,-11.1878583647923));
#120671=CARTESIAN_POINT('Ctrl Pts',(18.8573634539519,21.7067151227473,-11.3150341714737));
#120672=CARTESIAN_POINT('Ctrl Pts',(20.8992757606008,20.4581541188783,-11.4422099781552));
#120673=CARTESIAN_POINT('Ctrl Pts',(20.9546819490687,18.065406618053,-11.5693857848366));
#120674=CARTESIAN_POINT('Ctrl Pts',(18.9727502803322,16.7236699416198,-11.696561591518));
#120675=CARTESIAN_POINT('Ctrl Pts',(16.7717800479045,17.663904212636,-11.8237373981994));
#120676=CARTESIAN_POINT('Ctrl Pts',(16.371024832419,20.0235028449647,-11.9509132048809));
#120677=CARTESIAN_POINT('Ctrl Pts',(18.1381526704095,21.6376805466522,-12.0780890115623));
#120678=CARTESIAN_POINT('Ctrl Pts',(20.4519334508432,21.0255294635675,-12.2052648182438));
#120679=CARTESIAN_POINT('Ctrl Pts',(21.1896169171035,18.7486602200595,-12.3324406249252));
#120680=CARTESIAN_POINT('Ctrl Pts',(19.6744242746961,16.8959590286039,-12.4596164316066));
#120681=CARTESIAN_POINT('Ctrl Pts',(17.2964507295683,17.1671642407565,-12.5867922382881));
#120682=CARTESIAN_POINT('Ctrl Pts',(16.2373394156912,19.3134619072614,-12.7139680449695));
#120683=CARTESIAN_POINT('Ctrl Pts',(17.4687592276853,21.365757133357,-12.8411438516509));
#120684=CARTESIAN_POINT('Ctrl Pts',(19.8609589185792,21.4411964289083,-12.9683196583324));
#120685=CARTESIAN_POINT('Ctrl Pts',(21.2192437486358,19.4705689225376,-13.0954954650138));
#120686=CARTESIAN_POINT('Ctrl Pts',(20.2974716909424,17.2618030404029,-13.2226712716952));
#120687=CARTESIAN_POINT('Ctrl Pts',(17.9413113968065,16.8413043878911,-13.3498470783767));
#120688=CARTESIAN_POINT('Ctrl Pts',(16.3123936962972,18.5948543795921,-13.4770228850581));
#120689=CARTESIAN_POINT('Ctrl Pts',(16.9051494775971,20.9136797357071,-13.6041986917395));
#120690=CARTESIAN_POINT('Ctrl Pts',(19.1757621019364,21.6704021145338,-13.731374498421));
#120691=CARTESIAN_POINT('Ctrl Pts',(21.0410854165974,20.1707757009864,-13.8585503051024));
#120692=CARTESIAN_POINT('Ctrl Pts',(20.7898010554004,17.7906146521824,-13.9857261117838));
#120693=CARTESIAN_POINT('Ctrl Pts',(18.6524468232773,16.7135690009438,-14.1129019184653));
#120694=CARTESIAN_POINT('Ctrl Pts',(16.5899125690362,17.9277612832899,-14.2400777251467));
#120695=CARTESIAN_POINT('Ctrl Pts',(16.4944454556301,20.3192454414403,-14.3672535318281));
#120696=CARTESIAN_POINT('Ctrl Pts',(18.4536306342518,21.6939831925389,-14.4944293385096));
#120697=CARTESIAN_POINT('Ctrl Pts',(20.6700373042621,20.7907379758005,-14.621605145191));
#120698=CARTESIAN_POINT('Ctrl Pts',(21.1102499116389,18.438181215862,-14.7487809518724));
#120699=CARTESIAN_POINT('Ctrl Pts',(19.37040071179,16.7946377238266,-14.8759567585539));
#120700=CARTESIAN_POINT('Ctrl Pts',(17.0466933583566,17.3679566438234,-15.0031325652353));
#120701=CARTESIAN_POINT('Ctrl Pts',(16.27098512257,19.6321534509405,-15.1303083719167));
#120702=CARTESIAN_POINT('Ctrl Pts',(17.7549401648813,21.5099681065509,-15.2574841785982));
#120703=CARTESIAN_POINT('Ctrl Pts',(20.1371218386074,21.278622214454,-15.3846599852796));
#120704=CARTESIAN_POINT('Ctrl Pts',(21.2320263129741,19.1503612717033,-15.5118357919611));
#120705=CARTESIAN_POINT('Ctrl Pts',(20.0351466901858,17.0777325985008,-15.6390115986425));
#120706=CARTESIAN_POINT('Ctrl Pts',(17.6445457374235,16.9622443606664,-15.7661874053239));
#120707=CARTESIAN_POINT('Ctrl Pts',(16.2534514514175,18.9098498484046,-15.8933632120053));
#120708=CARTESIAN_POINT('Ctrl Pts',(17.1381064985295,21.1337419087451,-16.0205390186868));
#120709=CARTESIAN_POINT('Ctrl Pts',(19.4868947809189,21.5936376066338,-16.1477148253682));
#120710=CARTESIAN_POINT('Ctrl Pts',(21.1449488317356,19.8676111836039,-16.2748906320497));
#120711=CARTESIAN_POINT('Ctrl Pts',(20.5911069697954,17.5391847535037,-16.4020664387311));
#120712=CARTESIAN_POINT('Ctrl Pts',(18.3334847281261,16.7445450475071,-16.5292422454125));
#120713=CARTESIAN_POINT('Ctrl Pts',(16.4433103896197,18.2127246749636,-16.656418052094));
#120714=CARTESIAN_POINT('Ctrl Pts',(16.6547015924054,20.5967599531865,-16.7835938587754));
#120715=CARTESIAN_POINT('Ctrl Pts',(18.7737200283452,21.7094464843237,-16.9107696654568));
#120716=CARTESIAN_POINT('Ctrl Pts',(20.8562978035812,20.5299634371713,-17.0379454721383));
#120717=CARTESIAN_POINT('Ctrl Pts',(20.9917990686889,18.140413300518,-17.1651212788197));
#120718=CARTESIAN_POINT('Ctrl Pts',(19.0559098230889,16.7330600125345,-17.2922970855011));
#120719=CARTESIAN_POINT('Ctrl Pts',(16.8246882947818,17.5990628647505,-17.4194728921826));
#120720=CARTESIAN_POINT('Ctrl Pts',(16.3451417507631,19.9439179904547,-17.546648698864));
#120721=CARTESIAN_POINT('Ctrl Pts',(18.0572243811545,21.6163663499399,-17.6738245055454));
#120722=CARTESIAN_POINT('Ctrl Pts',(20.3902066364046,21.0820403772236,-17.8010003122269));
#120723=CARTESIAN_POINT('Ctrl Pts',(21.2037220985302,18.8311509882762,-17.9281761189083));
#120724=CARTESIAN_POINT('Ctrl Pts',(19.7514208234961,16.92874949148,-18.0553519255897));
#120725=CARTESIAN_POINT('Ctrl Pts',(17.3656990911611,17.1201711838414,-18.1825277322712));
#120726=CARTESIAN_POINT('Ctrl Pts',(16.2353085163561,19.229798543494,-18.3097035389526));
#120727=CARTESIAN_POINT('Ctrl Pts',(17.3973122915052,21.3221794063805,-18.4368793456341));
#120728=CARTESIAN_POINT('Ctrl Pts',(19.7856440750124,21.4776841982527,-18.5640551523154));
#120729=CARTESIAN_POINT('Ctrl Pts',(21.2091576920692,19.5536469249632,-18.6912309589969));
#120730=CARTESIAN_POINT('Ctrl Pts',(20.3618677523014,17.3152523642247,-18.8184067656783));
#120731=CARTESIAN_POINT('Ctrl Pts',(18.0211101865936,16.8160885976028,-18.9455825723598));
#120732=CARTESIAN_POINT('Ctrl Pts',(16.3343847778911,18.5141073945138,-19.0727583790412));
#120733=CARTESIAN_POINT('Ctrl Pts',(16.849157398292,20.8514819090936,-19.1999341857227));
#120734=CARTESIAN_POINT('Ctrl Pts',(19.093156119743,21.6838160799832,-19.327109992404));
#120735=CARTESIAN_POINT('Ctrl Pts',(21.0076513920927,20.2474950006713,-19.4542857990855));
#120736=CARTESIAN_POINT('Ctrl Pts',(20.8362126328065,17.8602540462332,-19.5814616057669));
#120737=CARTESIAN_POINT('Ctrl Pts',(18.7361242573121,16.7122387526989,-19.7086374124484));
#120738=CARTESIAN_POINT('Ctrl Pts',(16.6340870145935,17.8566816490089,-19.8358132191298));
#120739=CARTESIAN_POINT('Ctrl Pts',(16.4585895871711,20.243627889804,-19.9629890258113));
#120740=CARTESIAN_POINT('Ctrl Pts',(18.3706400116666,21.6832015249988,-20.0901648324927));
#120741=CARTESIAN_POINT('Ctrl Pts',(20.6160506226023,20.8546848763886,-20.2173406391741));
#120742=CARTESIAN_POINT('Ctrl Pts',(21.1347966972592,18.518187111326,-20.3445164458556));
#120743=CARTESIAN_POINT('Ctrl Pts',(19.4509606260352,16.8173065278623,-20.471692252537));
#120744=CARTESIAN_POINT('Ctrl Pts',(17.1093580392161,17.31248273928,-20.5988680592184));
#120745=CARTESIAN_POINT('Ctrl Pts',(16.2582629225594,19.5494468827994,-20.7260438658998));
#120746=CARTESIAN_POINT('Ctrl Pts',(17.6785042468215,21.475875836176,-20.8532196725813));
#120747=CARTESIAN_POINT('Ctrl Pts',(20.0670948425395,21.324481873539,-20.9803954792627));
#120748=CARTESIAN_POINT('Ctrl Pts',(21.2326586153631,19.2339836710777,-21.1075712859442));
#120749=CARTESIAN_POINT('Ctrl Pts',(20.1058486451417,17.1226225337713,-21.2347470926256));
#120750=CARTESIAN_POINT('Ctrl Pts',(17.7204710984363,16.9267880282744,-21.361922899307));
#120751=CARTESIAN_POINT('Ctrl Pts',(16.2649078451288,18.8274053200522,-21.4890987059885));
#120752=CARTESIAN_POINT('Ctrl Pts',(17.0746528024638,21.0783463863576,-21.6162745126699));
#120753=CARTESIAN_POINT('Ctrl Pts',(19.4066038595716,21.6192240457828,-21.7434503193513));
#120754=CARTESIAN_POINT('Ctrl Pts',(21.1220852841517,19.9442127979284,-21.8706447838074));
#120755=CARTESIAN_POINT('Ctrl Pts',(20.803831898832,18.3882311395412,-21.955447312703));
#120756=CARTESIAN_POINT('Ctrl Pts',(20.3504142092811,17.8498280795315,-21.997857906038));
#120757=CARTESIAN_POINT('Ctrl Pts',(18.0722627314315,16.7380050975816,1.38691141904346E-15));
#120758=CARTESIAN_POINT('Ctrl Pts',(17.9906109534297,16.7675693131061,-3.14694538653141E-14));
#120759=CARTESIAN_POINT('Ctrl Pts',(17.9108508876399,16.801533969706,6.86855221048143E-15));
#120760=CARTESIAN_POINT('Ctrl Pts',(17.833184560489,16.8395812357413,8.79504802320241E-16));
#120761=CARTESIAN_POINT('Ctrl Pts',(17.753672918112,16.8785324868355,-5.25183954169529E-15));
#120762=CARTESIAN_POINT('Ctrl Pts',(17.6763549684803,16.9217633043122,-1.85298947912786E-14));
#120763=CARTESIAN_POINT('Ctrl Pts',(17.601476924462,16.9689790985631,-1.06130382260261E-14));
#120764=CARTESIAN_POINT('Ctrl Pts',(17.5314114952683,17.0131602057527,-3.20501948859016E-15));
#120765=CARTESIAN_POINT('Ctrl Pts',(17.463482274071,17.0608314720442,1.11820055827351E-14));
#120766=CARTESIAN_POINT('Ctrl Pts',(17.3979218193959,17.1117790406503,1.23651089367627E-14));
#120767=CARTESIAN_POINT('Ctrl Pts',(17.3682534093495,17.1348346061396,1.26760648409614E-14));
#120768=CARTESIAN_POINT('Ctrl Pts',(17.3390705414607,17.1585614233309,2.36784452741916E-14));
#120769=CARTESIAN_POINT('Ctrl Pts',(17.310397157226,17.1829409553506,2.57155408078802E-14));
#120770=CARTESIAN_POINT('Ctrl Pts',(17.2926919353297,17.1979948122865,2.73538097927482E-14));
#120771=CARTESIAN_POINT('Ctrl Pts',(17.27518100039,17.2132975506653,1.30324840963727E-14));
#120772=CARTESIAN_POINT('Ctrl Pts',(17.257870302469,17.2288449191993,-8.4446338810551E-15));
#120773=CARTESIAN_POINT('Ctrl Pts',(17.2457082697189,17.239768083947,-2.37561771158851E-14));
#120774=CARTESIAN_POINT('Ctrl Pts',(17.2336433007629,17.2508137998582,-1.24432143521951E-14));
#120775=CARTESIAN_POINT('Ctrl Pts',(17.2216943574194,17.2619645032884,-7.15399961492835E-15));
#120776=CARTESIAN_POINT('Ctrl Pts',(17.1582625823413,17.3211587677193,2.03808243867262E-14));
#120777=CARTESIAN_POINT('Ctrl Pts',(17.0979931462804,17.3834003799274,6.45801759227035E-15));
#120778=CARTESIAN_POINT('Ctrl Pts',(17.041116608508,17.4484111431913,9.57567358739198E-15));
#120779=CARTESIAN_POINT('Ctrl Pts',(16.984962464847,17.5125961988015,1.26537319484047E-14));
#120780=CARTESIAN_POINT('Ctrl Pts',(16.9321151284108,17.5794813469685,1.14065042207504E-14));
#120781=CARTESIAN_POINT('Ctrl Pts',(16.8828390026402,17.6488249957258,1.34753319613878E-14));
#120782=CARTESIAN_POINT('Ctrl Pts',(16.8374017786391,17.7127663639311,1.53829857795583E-14));
#120783=CARTESIAN_POINT('Ctrl Pts',(16.7950011366565,17.7787988087843,-4.98584307276175E-15));
#120784=CARTESIAN_POINT('Ctrl Pts',(16.7558820673411,17.8467441370846,6.63358257213531E-15));
#120785=CARTESIAN_POINT('Ctrl Pts',(16.7395100185488,17.8751805045547,1.13870112004006E-14));
#120786=CARTESIAN_POINT('Ctrl Pts',(16.723713229623,17.903952012734,-1.077566553237E-15));
#120787=CARTESIAN_POINT('Ctrl Pts',(16.7085117731593,17.9330458325382,3.69149155687865E-15));
#120788=CARTESIAN_POINT('Ctrl Pts',(16.6986550833365,17.9519103905663,6.75998993358336E-15));
#120789=CARTESIAN_POINT('Ctrl Pts',(16.6890487140929,17.9709104592438,1.73723425931104E-14));
#120790=CARTESIAN_POINT('Ctrl Pts',(16.6796984374459,17.9900425446149,6.0507154842071E-15));
#120791=CARTESIAN_POINT('Ctrl Pts',(16.6737724856049,18.0021679416281,-6.19111889800206E-16));
#120792=CARTESIAN_POINT('Ctrl Pts',(16.6679532270762,18.0143385914813,2.13664567833998E-16));
#120793=CARTESIAN_POINT('Ctrl Pts',(16.6622433304787,18.0265499321002,2.5951463200613E-15));
#120794=CARTESIAN_POINT('Ctrl Pts',(16.6271177976284,18.1016703548131,1.76314342966372E-14));
#120795=CARTESIAN_POINT('Ctrl Pts',(16.5961057017263,18.1783725156421,-1.14329481650844E-14));
#120796=CARTESIAN_POINT('Ctrl Pts',(16.5694538401814,18.2564278430498,4.39925873507718E-15));
#120797=CARTESIAN_POINT('Ctrl Pts',(16.5428019786364,18.3344831704575,2.02314656352387E-14));
#120798=CARTESIAN_POINT('Ctrl Pts',(16.5205098793409,18.4138923942319,1.04011446651248E-14));
#120799=CARTESIAN_POINT('Ctrl Pts',(16.5028786483266,18.4944362051925,9.4091401336982E-15));
#120800=CARTESIAN_POINT('Ctrl Pts',(16.4850464602744,18.5758980374565,8.67831743648321E-15));
#120801=CARTESIAN_POINT('Ctrl Pts',(16.4719827280125,18.6585216956155,-2.53066140108434E-14));
#120802=CARTESIAN_POINT('Ctrl Pts',(16.4636117053936,18.7419152200439,-1.91235915991683E-14));
#120803=CARTESIAN_POINT('Ctrl Pts',(16.4601585345833,18.7763162839797,-1.6573003280011E-14));
#120804=CARTESIAN_POINT('Ctrl Pts',(16.4575045102803,18.8108481987005,-1.23100883047652E-14));
#120805=CARTESIAN_POINT('Ctrl Pts',(16.4556467292437,18.845482524778,-3.85802501057242E-15));
#120806=CARTESIAN_POINT('Ctrl Pts',(16.454914769638,18.859128335107,-7.53928088074055E-16));
#120807=CARTESIAN_POINT('Ctrl Pts',(16.4543064277075,18.8727920340357,-1.66414205223653E-14));
#120808=CARTESIAN_POINT('Ctrl Pts',(16.4538219965805,18.8864542247022,-1.65978342181461E-14));
#120809=CARTESIAN_POINT('Ctrl Pts',(16.4509322011605,18.9679538101119,-1.63169175235896E-14));
#120810=CARTESIAN_POINT('Ctrl Pts',(16.4524389841394,19.0495303086149,1.17186656710794E-14));
#120811=CARTESIAN_POINT('Ctrl Pts',(16.458209072107,19.1308246613079,1.11577413974828E-14));
#120812=CARTESIAN_POINT('Ctrl Pts',(16.4640075078908,19.212518404336,1.05940613637857E-14));
#120813=CARTESIAN_POINT('Ctrl Pts',(16.4741116098931,19.2939282562688,-2.01713604129673E-16));
#120814=CARTESIAN_POINT('Ctrl Pts',(16.4884373885337,19.3746780989613,-9.38138455808257E-15));
#120815=CARTESIAN_POINT('Ctrl Pts',(16.5025242207667,19.4540810770041,-1.84079434576874E-14));
#120816=CARTESIAN_POINT('Ctrl Pts',(16.5206935647272,19.5328467548947,8.94254489680765E-15));
#120817=CARTESIAN_POINT('Ctrl Pts',(16.5429083611757,19.6105921329322,6.30051566474776E-15));
#120818=CARTESIAN_POINT('Ctrl Pts',(16.5522119867773,19.6431521382056,5.19402563408715E-15));
#120819=CARTESIAN_POINT('Ctrl Pts',(16.5622256486948,19.6755328027596,3.88113245870864E-15));
#120820=CARTESIAN_POINT('Ctrl Pts',(16.5729486044555,19.7077040845634,4.66293670342566E-15));
#120821=CARTESIAN_POINT('Ctrl Pts',(16.5784892728338,19.7243273373082,5.05407298290637E-15));
#120822=CARTESIAN_POINT('Ctrl Pts',(16.5842201982241,19.7408967187103,-7.47574057736949E-15));
#120823=CARTESIAN_POINT('Ctrl Pts',(16.59013339505,19.757386717525,-3.5527136788005E-15));
#120824=CARTESIAN_POINT('Ctrl Pts',(16.6171691937068,19.8327808403536,1.42878117443501E-14));
#120825=CARTESIAN_POINT('Ctrl Pts',(16.6480432448069,19.9066161661436,5.97421475994626E-15));
#120826=CARTESIAN_POINT('Ctrl Pts',(16.6826949054327,19.9785209088995,-4.21884749357559E-15));
#120827=CARTESIAN_POINT('Ctrl Pts',(16.708683650902,20.0324494659664,-1.17360773291967E-14));
#120828=CARTESIAN_POINT('Ctrl Pts',(16.7367982565916,20.085291634914,2.01726906480219E-14));
#120829=CARTESIAN_POINT('Ctrl Pts',(16.7670276708943,20.1368764988564,7.7715611723761E-15));
#120830=CARTESIAN_POINT('Ctrl Pts',(16.776261941294,20.1526342828943,4.25330862624586E-15));
#120831=CARTESIAN_POINT('Ctrl Pts',(16.7856936339531,20.1682746431805,-1.0466123746905E-14));
#120832=CARTESIAN_POINT('Ctrl Pts',(16.7953226427023,20.1837924294014,-1.16573417585641E-15));
#120833=CARTESIAN_POINT('Ctrl Pts',(16.803547563051,20.1970474340419,6.67029465765244E-15));
#120834=CARTESIAN_POINT('Ctrl Pts',(16.8119141832479,20.2102092393014,-2.4083441391153E-14));
#120835=CARTESIAN_POINT('Ctrl Pts',(16.8204178931759,20.2232683327282,-1.87627691161651E-14));
#120836=CARTESIAN_POINT('Ctrl Pts',(16.8615694216389,20.2864644741072,6.85731831263342E-15));
#120837=CARTESIAN_POINT('Ctrl Pts',(16.9059580723631,20.3473056667748,2.60350180919675E-15));
#120838=CARTESIAN_POINT('Ctrl Pts',(16.9535504700224,20.4054521814502,-5.32907051820075E-15));
#120839=CARTESIAN_POINT('Ctrl Pts',(16.997682676699,20.459371171234,-1.13595455771569E-14));
#120840=CARTESIAN_POINT('Ctrl Pts',(17.0445702571952,20.51097318916,-3.05225759359301E-14));
#120841=CARTESIAN_POINT('Ctrl Pts',(17.0942091691994,20.55995417271,-1.27675647831893E-14));
#120842=CARTESIAN_POINT('Ctrl Pts',(17.0997977295932,20.5654686607127,-1.06144939056098E-14));
#120843=CARTESIAN_POINT('Ctrl Pts',(17.1054211843278,20.5709498884042,-1.65578075338009E-15));
#120844=CARTESIAN_POINT('Ctrl Pts',(17.1110791648801,20.5763977067475,-3.95239396766556E-14));
#120845=CARTESIAN_POINT('Ctrl Pts',(20.3504145393176,-17.5908279157877,
-0.0021418925797119));
#120846=CARTESIAN_POINT('Ctrl Pts',(20.8038322616566,-18.1292310654914,
-0.0445524841607392));
#120847=CARTESIAN_POINT('Ctrl Pts',(21.1220877448274,-19.685210814566,-0.129355011302244));
#120848=CARTESIAN_POINT('Ctrl Pts',(19.4066026967562,-21.3602255324577,
-0.256549474004229));
#120849=CARTESIAN_POINT('Ctrl Pts',(17.0746532893504,-20.819345744412,-0.383725280685663));
#120850=CARTESIAN_POINT('Ctrl Pts',(16.264907281043,-18.5684058059804,-0.510901087367098));
#120851=CARTESIAN_POINT('Ctrl Pts',(17.7204711810805,-16.6677874925037,
-0.638076894048532));
#120852=CARTESIAN_POINT('Ctrl Pts',(20.105848679288,-16.8636225373773,-0.765252700729966));
#120853=CARTESIAN_POINT('Ctrl Pts',(21.2326588952387,-18.9749835563125,
-0.8924285074114));
#120854=CARTESIAN_POINT('Ctrl Pts',(20.0670949402048,-21.0654821373604,
-1.01960431409284));
#120855=CARTESIAN_POINT('Ctrl Pts',(17.678504162672,-21.2168760062151,-1.14678012077427));
#120856=CARTESIAN_POINT('Ctrl Pts',(16.2582626864848,-19.2904469366441,
-1.2739559274557));
#120857=CARTESIAN_POINT('Ctrl Pts',(17.1093578926688,-17.0534825509078,
-1.40113173413714));
#120858=CARTESIAN_POINT('Ctrl Pts',(19.4509606903938,-16.5583063136444,
-1.52830754081857));
#120859=CARTESIAN_POINT('Ctrl Pts',(21.1347969203461,-18.2591870432273,
-1.65548334750001));
#120860=CARTESIAN_POINT('Ctrl Pts',(20.6160507961411,-20.5956850306546,
-1.78265915418144));
#120861=CARTESIAN_POINT('Ctrl Pts',(18.3706399783415,-21.4242017524251,
-1.90983496086288));
#120862=CARTESIAN_POINT('Ctrl Pts',(16.4585893765603,-19.9846279859987,
-2.03701076754431));
#120863=CARTESIAN_POINT('Ctrl Pts',(16.6340868204421,-17.5976815233674,
-2.16418657422575));
#120864=CARTESIAN_POINT('Ctrl Pts',(18.7361242574674,-16.453238521784,-2.29136238090717));
#120865=CARTESIAN_POINT('Ctrl Pts',(20.8362128272701,-17.6012539211848,
-2.41853818758862));
#120866=CARTESIAN_POINT('Ctrl Pts',(21.0076516023807,-19.9884950966021,
-2.54571399427004));
#120867=CARTESIAN_POINT('Ctrl Pts',(19.0931561529689,-21.4248163086708,
-2.67288980095148));
#120868=CARTESIAN_POINT('Ctrl Pts',(16.8491572239522,-20.5924820608467,
-2.80006560763291));
#120869=CARTESIAN_POINT('Ctrl Pts',(16.3343845559425,-18.2551073300457,
-2.92724141431435));
#120870=CARTESIAN_POINT('Ctrl Pts',(18.0211101206545,-16.557088376093,-3.05441722099578));
#120871=CARTESIAN_POINT('Ctrl Pts',(20.3618679028699,-17.0562521888763,
-3.18159302767722));
#120872=CARTESIAN_POINT('Ctrl Pts',(21.2091579210064,-19.2946469566574,
-3.30876883435865));
#120873=CARTESIAN_POINT('Ctrl Pts',(19.7856441722836,-21.2186844079067,
-3.43594464104009));
#120874=CARTESIAN_POINT('Ctrl Pts',(17.3973121678696,-21.0631796016525,
-3.56312044772152));
#120875=CARTESIAN_POINT('Ctrl Pts',(16.2353082852419,-18.9707985452326,
-3.69029625440296));
#120876=CARTESIAN_POINT('Ctrl Pts',(17.3656989646013,-16.8611709904523,
-3.81747206108439));
#120877=CARTESIAN_POINT('Ctrl Pts',(19.7514209176014,-16.6697492803852,
-3.94464786776582));
#120878=CARTESIAN_POINT('Ctrl Pts',(21.2037223269647,-18.5721509531424,
-4.07182367444726));
#120879=CARTESIAN_POINT('Ctrl Pts',(20.390206789594,-20.8230405502836,-4.19899948112869));
#120880=CARTESIAN_POINT('Ctrl Pts',(18.0572243185569,-21.357366572422,-4.32617528781012));
#120881=CARTESIAN_POINT('Ctrl Pts',(16.3451415298078,-19.6849180582454,
-4.45335109449157));
#120882=CARTESIAN_POINT('Ctrl Pts',(16.8246881181817,-17.340062715656,-4.58052690117299));
#120883=CARTESIAN_POINT('Ctrl Pts',(19.0559098528636,-16.4740597833398,
-4.70770270785444));
#120884=CARTESIAN_POINT('Ctrl Pts',(20.9917992775219,-17.8814132014949,
-4.83487851453586));
#120885=CARTESIAN_POINT('Ctrl Pts',(20.8562979998813,-20.2709635591674,
-4.9620543212173));
#120886=CARTESIAN_POINT('Ctrl Pts',(18.7737200320192,-21.4504467154151,
-5.08923012789874));
#120887=CARTESIAN_POINT('Ctrl Pts',(16.6547014000827,-20.3377600813612,
-5.21640593458017));
#120888=CARTESIAN_POINT('Ctrl Pts',(16.4433101777445,-17.9537245826292,
-5.34358174126161));
#120889=CARTESIAN_POINT('Ctrl Pts',(18.3334846910807,-16.4855448193747,
-5.47075754794303));
#120890=CARTESIAN_POINT('Ctrl Pts',(20.5911071415668,-17.2801845988705,
-5.59793335462448));
#120891=CARTESIAN_POINT('Ctrl Pts',(21.144949054734,-19.6086112443364,-5.7251091613059));
#120892=CARTESIAN_POINT('Ctrl Pts',(19.4868948505574,-21.3346378270135,
-5.85228496798734));
#120893=CARTESIAN_POINT('Ctrl Pts',(17.1381063509189,-20.8747420865874,
-5.97946077466877));
#120894=CARTESIAN_POINT('Ctrl Pts',(16.2534512219814,-18.6508498205501,
-6.10663658135021));
#120895=CARTESIAN_POINT('Ctrl Pts',(17.6445456366553,-16.7032441526699,
-6.23381238803165));
#120896=CARTESIAN_POINT('Ctrl Pts',(20.0351468105341,-16.8187324011862,
-6.36098819471307));
#120897=CARTESIAN_POINT('Ctrl Pts',(21.2320265440266,-18.8913612660945,
-6.48816400139451));
#120898=CARTESIAN_POINT('Ctrl Pts',(20.137121968388,-21.0196224056966,-6.61533980807595));
#120899=CARTESIAN_POINT('Ctrl Pts',(17.7549400743241,-21.2509683191918,
-6.74251561475738));
#120900=CARTESIAN_POINT('Ctrl Pts',(16.2709848947557,-19.3731534898947,
-6.86969142143882));
#120901=CARTESIAN_POINT('Ctrl Pts',(17.0466932022907,-17.1089564733528,
-6.99686722812024));
#120902=CARTESIAN_POINT('Ctrl Pts',(19.3704007706532,-16.5356375003274,
-7.12404303480169));
#120903=CARTESIAN_POINT('Ctrl Pts',(21.1102501314279,-18.1791811443807,
-7.25121884148312));
#120904=CARTESIAN_POINT('Ctrl Pts',(20.6700374833341,-20.5317381219169,
-7.37839464816456));
#120905=CARTESIAN_POINT('Ctrl Pts',(18.4536306083194,-21.4349834222001,
-7.50557045484598));
#120906=CARTESIAN_POINT('Ctrl Pts',(16.4944452484846,-20.0602455439464,
-7.63274626152742));
#120907=CARTESIAN_POINT('Ctrl Pts',(16.5899123707208,-17.668761164598,-7.75992206820886));
#120908=CARTESIAN_POINT('Ctrl Pts',(18.6524468157339,-16.4545687699462,
-7.88709787489029));
#120909=CARTESIAN_POINT('Ctrl Pts',(20.7898012455497,-17.531614520805,-8.01427368157173));
#120910=CARTESIAN_POINT('Ctrl Pts',(21.0410856299891,-19.9117757897599,
-8.14144948825315));
#120911=CARTESIAN_POINT('Ctrl Pts',(19.175762142797,-21.4114023420139,-8.2686252949346));
#120912=CARTESIAN_POINT('Ctrl Pts',(16.9051493084394,-20.6546798931949,
-8.39580110161602));
#120913=CARTESIAN_POINT('Ctrl Pts',(16.312393472313,-18.3358543226023,-8.52297690829747));
#120914=CARTESIAN_POINT('Ctrl Pts',(17.9413113234874,-16.5823041687085,
-8.65015271497889));
#120915=CARTESIAN_POINT('Ctrl Pts',(20.2974718355542,-17.0028028601137,
-8.77732852166034));
#120916=CARTESIAN_POINT('Ctrl Pts',(21.2192439785061,-19.211568946546,-8.90450432834176));
#120917=CARTESIAN_POINT('Ctrl Pts',(19.8609590228163,-21.1821966351882,
-9.0316801350232));
#120918=CARTESIAN_POINT('Ctrl Pts',(17.4687591106581,-21.1067573326593,
-9.15885594170464));
#120919=CARTESIAN_POINT('Ctrl Pts',(16.2373391847649,-19.0544619167386,
-9.28603174838607));
#120920=CARTESIAN_POINT('Ctrl Pts',(17.2964505966034,-16.908164051714,-9.4132075550675));
#120921=CARTESIAN_POINT('Ctrl Pts',(19.6744243616797,-16.6369588144763,
-9.54038336174894));
#120922=CARTESIAN_POINT('Ctrl Pts',(21.1896171442334,-18.4896601772957,
-9.66755916843036));
#120923=CARTESIAN_POINT('Ctrl Pts',(20.4519336097419,-20.7665296314006,
-9.79473497511181));
#120924=CARTESIAN_POINT('Ctrl Pts',(18.1381526152972,-21.3786807711059,
-9.92191078179324));
#120925=CARTESIAN_POINT('Ctrl Pts',(16.3710246138578,-19.7645029201165,
-10.0490865884747));
#120926=CARTESIAN_POINT('Ctrl Pts',(16.7717798664108,-17.4049040695389,
-10.1762623951561));
#120927=CARTESIAN_POINT('Ctrl Pts',(18.9727503024152,-16.4646697115565,
-10.3034382018376));
#120928=CARTESIAN_POINT('Ctrl Pts',(20.9546821544686,-17.8064065120923,
-10.430614008519));
#120929=CARTESIAN_POINT('Ctrl Pts',(20.8992759608759,-20.1991542342326,
-10.5577898152005));
#120930=CARTESIAN_POINT('Ctrl Pts',(18.8573634653625,-21.4477153535862,
-10.6849656218819));
#120931=CARTESIAN_POINT('Ctrl Pts',(16.702272647179,-20.4066125375889,-10.8121414285633));
#120932=CARTESIAN_POINT('Ctrl Pts',(16.4111655719875,-18.0309930017901,
-10.9393172352448));
#120933=CARTESIAN_POINT('Ctrl Pts',(18.2511149131333,-16.5003402227076,
-11.0664930419262));
#120934=CARTESIAN_POINT('Ctrl Pts',(20.5340813502507,-17.2189331221239,
-11.1936688486076));
#120935=CARTESIAN_POINT('Ctrl Pts',(21.165584874162,-19.5275073157298,-11.3208446552891));
#120936=CARTESIAN_POINT('Ctrl Pts',(19.5662601972076,-21.3080892671662,
-11.4480204619705));
#120937=CARTESIAN_POINT('Ctrl Pts',(17.2033884452088,-20.9271055513698,
-11.575196268652));
#120938=CARTESIAN_POINT('Ctrl Pts',(16.2447577942637,-18.7340850810675,
-11.7023720753333));
#120939=CARTESIAN_POINT('Ctrl Pts',(17.5698523672862,-16.7409880235606,
-11.8295478820148));
#120940=CARTESIAN_POINT('Ctrl Pts',(19.9629801381724,-16.7763572235568,
-11.9567236886962));
#120941=CARTESIAN_POINT('Ctrl Pts',(21.2285949113957,-18.8077436353198,
-12.0838994953777));
#120942=CARTESIAN_POINT('Ctrl Pts',(20.2055736854352,-20.9714763081171,
-12.2110753020591));
#120943=CARTESIAN_POINT('Ctrl Pts',(17.8324749392518,-21.2824648110527,
-12.3382511087405));
#120944=CARTESIAN_POINT('Ctrl Pts',(16.2864694813489,-19.4553964948066,
-12.465426915422));
#120945=CARTESIAN_POINT('Ctrl Pts',(16.985921363432,-17.1664931388855,-12.5926027221034));
#120946=CARTESIAN_POINT('Ctrl Pts',(19.2891268965698,-16.515681506983,-12.7197785287849));
#120947=CARTESIAN_POINT('Ctrl Pts',(21.0830379571657,-18.100040877444,-12.8469543354662));
#120948=CARTESIAN_POINT('Ctrl Pts',(20.7218524898006,-20.4660198643034,
-12.9741301421477));
#120949=CARTESIAN_POINT('Ctrl Pts',(18.5369357430837,-21.4429795963352,
-13.1013059488291));
#120950=CARTESIAN_POINT('Ctrl Pts',(16.5328132209002,-20.1346201563596,
-13.2284817555106));
#120951=CARTESIAN_POINT('Ctrl Pts',(16.5481429474813,-17.7412801246093,
-13.355657562192));
#120952=CARTESIAN_POINT('Ctrl Pts',(18.5688608501589,-16.4587004327796,
-13.4828333688734));
#120953=CARTESIAN_POINT('Ctrl Pts',(20.7410836731242,-17.4635683422508,
-13.6100091755549));
#120954=CARTESIAN_POINT('Ctrl Pts',(21.0719317996599,-19.8339799152194,
-13.7371849822363));
#120955=CARTESIAN_POINT('Ctrl Pts',(19.2578726084204,-21.3952296578215,
-13.8643607889177));
#120956=CARTESIAN_POINT('Ctrl Pts',(16.9631928141561,-20.7149678333072,
-13.9915365955992));
#120957=CARTESIAN_POINT('Ctrl Pts',(16.2931187042143,-18.4172924438578,
-14.1187124022806));
#120958=CARTESIAN_POINT('Ctrl Pts',(17.8624016849767,-16.6101780494751,
-14.245888208962));
#120959=CARTESIAN_POINT('Ctrl Pts',(20.2313220222805,-16.9515399448363,
-14.3730640156435));
#120960=CARTESIAN_POINT('Ctrl Pts',(21.2265423384276,-19.1281997782562,
-14.5002398223249));
#120961=CARTESIAN_POINT('Ctrl Pts',(19.9350097636923,-21.1432072513177,
-14.6274156290064));
#120962=CARTESIAN_POINT('Ctrl Pts',(17.5416252738421,-21.1479180729553,
-14.7545914356878));
#120963=CARTESIAN_POINT('Ctrl Pts',(16.2421705881198,-19.1380103567032,
-14.8817672423692));
#120964=CARTESIAN_POINT('Ctrl Pts',(17.2288147274218,-16.9574496832805,
-15.0089430490507));
#120965=CARTESIAN_POINT('Ctrl Pts',(19.5963729319801,-16.6067651296939,
-15.1361188557321));
#120966=CARTESIAN_POINT('Ctrl Pts',(21.1727574963474,-18.4076880079206,
-15.2632946624135));
#120967=CARTESIAN_POINT('Ctrl Pts',(20.511733424177,-20.707983355068,-15.3904704690949));
#120968=CARTESIAN_POINT('Ctrl Pts',(18.2197492739044,-21.397272962559,-15.5176462757764));
#120969=CARTESIAN_POINT('Ctrl Pts',(16.3995582468247,-19.8431763976587,
-15.6448220824578));
#120970=CARTESIAN_POINT('Ctrl Pts',(16.7210726364874,-17.471480800552,-15.7719978891392));
#120971=CARTESIAN_POINT('Ctrl Pts',(18.8893229458104,-16.4580696775538,
-15.8991736958207));
#120972=CARTESIAN_POINT('Ctrl Pts',(20.9150740927816,-17.732684834627,-16.0263495025021));
#120973=CARTESIAN_POINT('Ctrl Pts',(20.939825132351,-20.1259459766957,-16.1535253091836));
#120974=CARTESIAN_POINT('Ctrl Pts',(18.9408685219365,-21.4421845484509,
-16.280701115865));
#120975=CARTESIAN_POINT('Ctrl Pts',(16.7521228823537,-20.4738333552863,
-16.4078769225464));
#120976=CARTESIAN_POINT('Ctrl Pts',(16.3816264890446,-18.1092945142771,
-16.5350527292279));
#120977=CARTESIAN_POINT('Ctrl Pts',(18.1692867872707,-16.5178856522175,
-16.6622285359093));
#120978=CARTESIAN_POINT('Ctrl Pts',(20.475036408121,-17.1596256260733,-16.7894043425907));
#120979=CARTESIAN_POINT('Ctrl Pts',(21.1834931854267,-19.445757840707,-16.9165801492722));
#120980=CARTESIAN_POINT('Ctrl Pts',(19.6446919977966,-21.2788978825597,
-17.0437559559536));
#120981=CARTESIAN_POINT('Ctrl Pts',(17.2703874261082,-20.9772535407345,
-17.1709317626351));
#120982=CARTESIAN_POINT('Ctrl Pts',(16.2388565489241,-18.8175647766965,
-17.2981075693165));
#120983=CARTESIAN_POINT('Ctrl Pts',(17.4964649220338,-16.7812119860486,
-17.4252833759979));
#120984=CARTESIAN_POINT('Ctrl Pts',(19.8894349190882,-16.7364224639015,
-17.5524591826793));
#120985=CARTESIAN_POINT('Ctrl Pts',(21.2223650922577,-18.7242878168747,
-17.6796349893608));
#120986=CARTESIAN_POINT('Ctrl Pts',(20.2723747386373,-20.9210649644522,
-17.8068107960422));
#120987=CARTESIAN_POINT('Ctrl Pts',(17.9110210446204,-21.3113472211018,
-17.9339866027237));
#120988=CARTESIAN_POINT('Ctrl Pts',(16.3046994623321,-19.5370748399901,
-18.061162409405));
#120989=CARTESIAN_POINT('Ctrl Pts',(16.9271103439532,-17.226032607035,-18.1883382160865));
#120990=CARTESIAN_POINT('Ctrl Pts',(19.2072303367862,-16.498458331493,-18.3155140227679));
#120991=CARTESIAN_POINT('Ctrl Pts',(21.0531908675876,-18.0218562528634,
-18.4426898294494));
#120992=CARTESIAN_POINT('Ctrl Pts',(20.7714377226303,-20.3986033309466,
-18.5698656361308));
#120993=CARTESIAN_POINT('Ctrl Pts',(18.6204619247414,-21.4481816393175,
-18.6970414428122));
#120994=CARTESIAN_POINT('Ctrl Pts',(16.57365026406,-20.2076682239227,-18.8242172494937));
#120995=CARTESIAN_POINT('Ctrl Pts',(16.508825399435,-17.8151571490185,-18.9513930561751));
#120996=CARTESIAN_POINT('Ctrl Pts',(18.4854601213826,-16.4656288287323,
-19.0785688628566));
#120997=CARTESIAN_POINT('Ctrl Pts',(20.6901147549395,-17.3971917378963,
-19.205744669538));
#120998=CARTESIAN_POINT('Ctrl Pts',(21.1001555127428,-19.7551947225373,
-19.3329204762194));
#120999=CARTESIAN_POINT('Ctrl Pts',(19.3393954444469,-21.3763164063757,
-19.4600962829008));
#121000=CARTESIAN_POINT('Ctrl Pts',(17.0232226373686,-20.7732782473175,
-19.5872720895823));
#121001=CARTESIAN_POINT('Ctrl Pts',(16.2765818653196,-18.4993303570677,
-19.7144478962637));
#121002=CARTESIAN_POINT('Ctrl Pts',(17.784469731095,-16.6406787308973,-19.8416237029452));
#121003=CARTESIAN_POINT('Ctrl Pts',(20.1634926381912,-16.9025209845322,
-19.9687995096266));
#121004=CARTESIAN_POINT('Ctrl Pts',(21.2310448625075,-19.0446328907795,
-20.095975316308));
#121005=CARTESIAN_POINT('Ctrl Pts',(20.0077132391621,-21.1017601371114,
-20.2231511229895));
#121006=CARTESIAN_POINT('Ctrl Pts',(17.6158291027325,-21.1866153706034,
-20.3503269296709));
#121007=CARTESIAN_POINT('Ctrl Pts',(16.2497967305417,-19.2213506919733,
-20.4775027363524));
#121008=CARTESIAN_POINT('Ctrl Pts',(17.162867889616,-17.0089715551397,-20.6046785430338));
#121009=CARTESIAN_POINT('Ctrl Pts',(19.517352896747,-16.5792041101631,-20.7318543497152));
#121010=CARTESIAN_POINT('Ctrl Pts',(21.1531647647671,-18.3263225093304,
-20.8590301563966));
#121011=CARTESIAN_POINT('Ctrl Pts',(20.5695343966717,-20.6474748753932,
-20.9862059630781));
#121012=CARTESIAN_POINT('Ctrl Pts',(18.3019319358899,-21.4131078753525,
-21.1133817697595));
#121013=CARTESIAN_POINT('Ctrl Pts',(16.4306927582234,-19.9208780183908,
-21.2405575764409));
#121014=CARTESIAN_POINT('Ctrl Pts',(16.672657339533,-17.5396647158853,-21.3677333831224));
#121015=CARTESIAN_POINT('Ctrl Pts',(18.8056557936095,-16.4543701890598,
-21.4949091898038));
#121016=CARTESIAN_POINT('Ctrl Pts',(20.8731458592265,-17.6601321897591,
-21.6220849964852));
#121017=CARTESIAN_POINT('Ctrl Pts',(20.9776565367662,-20.0518039395808,
-21.7492608031667));
#121018=CARTESIAN_POINT('Ctrl Pts',(19.0246114636561,-21.4331200318623,
-21.8764366098481));
#121019=CARTESIAN_POINT('Ctrl Pts',(16.8032831871667,-20.5407974041735,
-22.0036124165295));
#121020=CARTESIAN_POINT('Ctrl Pts',(16.3565571918356,-18.1855239713029,
-22.130788223211));
#121021=CARTESIAN_POINT('Ctrl Pts',(17.5080922582077,-17.0924952631291,
-22.2155720943319));
#121022=CARTESIAN_POINT('Ctrl Pts',(18.187758323454,-16.9106265641217,-22.2579640298924));
#121023=CARTESIAN_POINT('Ctrl Pts',(20.4651728847368,-17.4941906656173,
0.0844764971292257));
#121024=CARTESIAN_POINT('Ctrl Pts',(20.9507812774351,-18.0708180784204,
0.0420659055481983));
#121025=CARTESIAN_POINT('Ctrl Pts',(21.2916315045783,-19.7372655677721,
-0.0427366215933074));
#121026=CARTESIAN_POINT('Ctrl Pts',(19.454354539323,-21.53119898684,-0.16993108429529));
#121027=CARTESIAN_POINT('Ctrl Pts',(16.9568469479949,-20.951919105231,-0.297106890976726));
#121028=CARTESIAN_POINT('Ctrl Pts',(16.0896125232803,-18.5411723000033,
-0.424282697658159));
#121029=CARTESIAN_POINT('Ctrl Pts',(17.648515078568,-16.5056184191814,-0.551458504339595));
#121030=CARTESIAN_POINT('Ctrl Pts',(20.2032439208991,-16.7153568936381,
-0.678634311021027));
#121031=CARTESIAN_POINT('Ctrl Pts',(21.41005272189,-18.9766152880434,-0.805810117702463));
#121032=CARTESIAN_POINT('Ctrl Pts',(20.1617388362496,-21.2155301029391,
-0.932985924383897));
#121033=CARTESIAN_POINT('Ctrl Pts',(17.6035685858491,-21.3776722727239,
-1.06016173106533));
#121034=CARTESIAN_POINT('Ctrl Pts',(16.0824961916403,-19.3144751852875,
-1.18733753774677));
#121035=CARTESIAN_POINT('Ctrl Pts',(16.9940154259929,-16.918696135723,-1.3145133444282));
#121036=CARTESIAN_POINT('Ctrl Pts',(19.5018617560294,-16.3883645566231,
-1.44168915110964));
#121037=CARTESIAN_POINT('Ctrl Pts',(21.3052429758379,-18.2100003608074,
-1.56886495779107));
#121038=CARTESIAN_POINT('Ctrl Pts',(20.7496681511615,-20.7123794613962,
-1.69604076447251));
#121039=CARTESIAN_POINT('Ctrl Pts',(18.344843009889,-21.599717237933,-1.82321657115394));
#121040=CARTESIAN_POINT('Ctrl Pts',(16.2970451984157,-20.057940045637,-1.95039237783538));
#121041=CARTESIAN_POINT('Ctrl Pts',(16.4850021913768,-17.5015308492868,
-2.07756818451681));
#121042=CARTESIAN_POINT('Ctrl Pts',(18.7362750704342,-16.275837412191,-2.20474399119824));
#121043=CARTESIAN_POINT('Ctrl Pts',(20.9854607212405,-17.5053568716867,
-2.33191979787968));
#121044=CARTESIAN_POINT('Ctrl Pts',(21.1690708977422,-20.0620817041385,
-2.45909560456111));
#121045=CARTESIAN_POINT('Ctrl Pts',(19.1186546651756,-21.6003754249779,
-2.58627141124255));
#121046=CARTESIAN_POINT('Ctrl Pts',(16.7153416505994,-20.7089490947747,
-2.71344721792398));
#121047=CARTESIAN_POINT('Ctrl Pts',(16.1640223800872,-18.2056310058767,
-2.84062302460542));
#121048=CARTESIAN_POINT('Ctrl Pts',(17.9704980647556,-16.3870601508454,
-2.96779883128685));
#121049=CARTESIAN_POINT('Ctrl Pts',(20.477439386886,-16.9216624058443,-3.09497463796828));
#121050=CARTESIAN_POINT('Ctrl Pts',(21.3848832815229,-19.3189733883075,
-3.22215044464972));
#121051=CARTESIAN_POINT('Ctrl Pts',(19.8603062977751,-21.3796090630069,
-3.34932625133115));
#121052=CARTESIAN_POINT('Ctrl Pts',(17.3024131922505,-21.213064097291,-3.47650205801259));
#121053=CARTESIAN_POINT('Ctrl Pts',(16.0579121285487,-18.9721331595253,
-3.60367786469402));
#121054=CARTESIAN_POINT('Ctrl Pts',(17.2685555901523,-16.7127312976299,
-3.73085367137545));
#121055=CARTESIAN_POINT('Ctrl Pts',(19.8236533420561,-16.5077194854014,
-3.85802947805689));
#121056=CARTESIAN_POINT('Ctrl Pts',(21.3790617841357,-18.5451833361938,
-3.98520528473832));
#121057=CARTESIAN_POINT('Ctrl Pts',(20.5077902103209,-20.9558762261203,
-4.11238109141976));
#121058=CARTESIAN_POINT('Ctrl Pts',(18.009176212373,-21.5281370531764,-4.23955689810119));
#121059=CARTESIAN_POINT('Ctrl Pts',(16.1755430519351,-19.7369520270363,
-4.36673270478263));
#121060=CARTESIAN_POINT('Ctrl Pts',(16.6891353455995,-17.2256222357103,
-4.49390851146406));
#121061=CARTESIAN_POINT('Ctrl Pts',(19.0787640410623,-16.2981368920303,
-4.6210843181455));
#121062=CARTESIAN_POINT('Ctrl Pts',(21.15209312732,-17.805406232592,-4.74826012482693));
#121063=CARTESIAN_POINT('Ctrl Pts',(21.0069718530473,-20.364604189115,-4.87543593150836));
#121064=CARTESIAN_POINT('Ctrl Pts',(18.7765399801474,-21.6278254782292,
-5.0026117381898));
#121065=CARTESIAN_POINT('Ctrl Pts',(16.5070803157911,-20.4361429715275,
-5.12978754487123));
#121066=CARTESIAN_POINT('Ctrl Pts',(16.2806812434728,-17.8828514047509,
-5.25696335155267));
#121067=CARTESIAN_POINT('Ctrl Pts',(18.3050498601331,-16.3104373152697,
-5.38413915823409));
#121068=CARTESIAN_POINT('Ctrl Pts',(20.7229536064731,-17.1614930351577,
-5.51131496491554));
#121069=CARTESIAN_POINT('Ctrl Pts',(21.3161158672572,-19.6552277638931,
-5.63849077159696));
#121070=CARTESIAN_POINT('Ctrl Pts',(19.5403470840179,-21.503794666494,-5.76566657827842));
#121071=CARTESIAN_POINT('Ctrl Pts',(17.0248048987365,-21.0112483448259,
-5.89284238495983));
#121072=CARTESIAN_POINT('Ctrl Pts',(16.0773431342523,-18.6294694781468,
-6.02001819164128));
#121073=CARTESIAN_POINT('Ctrl Pts',(17.5671991533703,-16.5435923467661,
-6.1471939983227));
#121074=CARTESIAN_POINT('Ctrl Pts',(20.127522529443,-16.6672797545901,-6.27436980500414));
#121075=CARTESIAN_POINT('Ctrl Pts',(21.4093754765144,-18.8870561818465,
-6.40154561168558));
#121076=CARTESIAN_POINT('Ctrl Pts',(20.2367374764131,-21.1664145313908,
-6.52872141836701));
#121077=CARTESIAN_POINT('Ctrl Pts',(17.6854311121095,-21.4141849904505,
-6.65589722504845));
#121078=CARTESIAN_POINT('Ctrl Pts',(16.0961216209204,-19.4030535412072,
-6.78307303172988));
#121079=CARTESIAN_POINT('Ctrl Pts',(16.9269018173399,-16.9781084634466,
-6.91024883841132));
#121080=CARTESIAN_POINT('Ctrl Pts',(19.4155824351873,-16.3640863569478,
-7.03742464509275));
#121081=CARTESIAN_POINT('Ctrl Pts',(21.2789534725274,-18.1243143939139,
-7.16460045177418));
#121082=CARTESIAN_POINT('Ctrl Pts',(20.8074876564503,-20.6438926025015,
-7.29177625845562));
#121083=CARTESIAN_POINT('Ctrl Pts',(18.4337256107381,-21.6112643589919,
-7.41895206513705));
#121084=CARTESIAN_POINT('Ctrl Pts',(16.3354466800433,-20.1389261186678,
-7.54612787181849));
#121085=CARTESIAN_POINT('Ctrl Pts',(16.4376915494001,-17.5776568334092,
-7.67330367849992));
#121086=CARTESIAN_POINT('Ctrl Pts',(18.646656897206,-16.2772621021406,-7.80047948518135));
#121087=CARTESIAN_POINT('Ctrl Pts',(20.9357541207011,-17.4307733792013,
-7.92765529186279));
#121088=CARTESIAN_POINT('Ctrl Pts',(21.2048785947256,-19.9799156628723,
-8.05483109854422));
#121089=CARTESIAN_POINT('Ctrl Pts',(19.2071253181107,-21.5860091254994,
-8.18200690522566));
#121090=CARTESIAN_POINT('Ctrl Pts',(16.7753089275983,-20.7755627005247,
-8.3091827119071));
#121091=CARTESIAN_POINT('Ctrl Pts',(16.1404700259359,-18.2921106808846,
-8.43635851858852));
#121092=CARTESIAN_POINT('Ctrl Pts',(17.8850339028528,-16.4140661541825,
-8.56353432526996));
#121093=CARTESIAN_POINT('Ctrl Pts',(20.4084714811236,-16.8644184090784,
-8.69071013195139));
#121094=CARTESIAN_POINT('Ctrl Pts',(21.3956854048846,-19.2299972037186,
-8.81788593863284));
#121095=CARTESIAN_POINT('Ctrl Pts',(19.9409681724916,-21.3405308183994,
-8.94506174531426));
#121096=CARTESIAN_POINT('Ctrl Pts',(17.3789325547309,-21.2597356561407,
-9.0722375519957));
#121097=CARTESIAN_POINT('Ctrl Pts',(16.0600872130337,-19.0617362636016,
-9.19941335867713));
#121098=CARTESIAN_POINT('Ctrl Pts',(17.1943908916334,-16.7630606602087,
-9.32658916535856));
#121099=CARTESIAN_POINT('Ctrl Pts',(19.7411903682412,-16.4726010401766,
-9.45376497204));
#121100=CARTESIAN_POINT('Ctrl Pts',(21.3639551952721,-18.4568360769276,
-9.58094077872143));
#121101=CARTESIAN_POINT('Ctrl Pts',(20.5738993640695,-20.8953532797583,
-9.70811658540287));
#121102=CARTESIAN_POINT('Ctrl Pts',(18.0958500633667,-21.5509644665186,
-9.83529239208431));
#121103=CARTESIAN_POINT('Ctrl Pts',(16.2032637214729,-19.8221870651751,
-9.96246819876573));
#121104=CARTESIAN_POINT('Ctrl Pts',(16.6324708399194,-17.2950670414339,
-10.0896440054472));
#121105=CARTESIAN_POINT('Ctrl Pts',(18.9897005271298,-16.2880801663194,
-10.2168198121286));
#121106=CARTESIAN_POINT('Ctrl Pts',(21.1123408512631,-17.7250743970949,
-10.3439956188101));
#121107=CARTESIAN_POINT('Ctrl Pts',(21.0530010608437,-20.2876967169446,
-10.4711714254915));
#121108=CARTESIAN_POINT('Ctrl Pts',(18.8661217305387,-21.6249002016856,
-10.598347232173));
#121109=CARTESIAN_POINT('Ctrl Pts',(16.5580289128638,-20.5098836502765,
-10.7255230388544));
#121110=CARTESIAN_POINT('Ctrl Pts',(16.2462545116391,-17.965605542903,-10.8526988455358));
#121111=CARTESIAN_POINT('Ctrl Pts',(18.2168321890867,-16.3262831273715,
-10.9798746522173));
#121112=CARTESIAN_POINT('Ctrl Pts',(20.6618792339927,-17.0958929721078,
-11.1070504588987));
#121113=CARTESIAN_POINT('Ctrl Pts',(21.3382167393905,-19.5683658119407,
-11.2342262655802));
#121114=CARTESIAN_POINT('Ctrl Pts',(19.6253470223175,-21.4753612752947,
-11.3614020722615));
#121115=CARTESIAN_POINT('Ctrl Pts',(17.0947217355035,-21.0673293860297,
-11.488577878943));
#121116=CARTESIAN_POINT('Ctrl Pts',(16.0680325112813,-18.7186140772312,
-11.6157536856244));
#121117=CARTESIAN_POINT('Ctrl Pts',(17.4872029893547,-16.584015867009,-11.7429294923059));
#121118=CARTESIAN_POINT('Ctrl Pts',(20.0502323397452,-16.6218961251351,
-11.8701052989873));
#121119=CARTESIAN_POINT('Ctrl Pts',(21.4057002130119,-18.797502065893,-11.9972811056688));
#121120=CARTESIAN_POINT('Ctrl Pts',(20.3100489652568,-21.1148502719707,
-12.1244569123501));
#121121=CARTESIAN_POINT('Ctrl Pts',(17.7684706125095,-21.4479175951428,
-12.2516327190316));
#121122=CARTESIAN_POINT('Ctrl Pts',(16.1127055452724,-19.4911354388884,
-12.378808525713));
#121123=CARTESIAN_POINT('Ctrl Pts',(16.8618154443651,-17.0397299799731,
-12.5059843323945));
#121124=CARTESIAN_POINT('Ctrl Pts',(19.3285384723745,-16.3427135755694,
-12.6331601390759));
#121125=CARTESIAN_POINT('Ctrl Pts',(21.2498093531994,-18.0395555150007,
-12.7603359457573));
#121126=CARTESIAN_POINT('Ctrl Pts',(20.8629813012026,-20.5735086367272,
-12.8875117524388));
#121127=CARTESIAN_POINT('Ctrl Pts',(18.5229450448345,-21.6198282264327,
-13.0146875591202));
#121128=CARTESIAN_POINT('Ctrl Pts',(16.3765386102829,-20.2185810024805,
-13.1418633658017));
#121129=CARTESIAN_POINT('Ctrl Pts',(16.3929566802409,-17.6553243216352,
-13.2690391724831));
#121130=CARTESIAN_POINT('Ctrl Pts',(18.5571366945425,-16.2816870949206,
-13.3962149791645));
#121131=CARTESIAN_POINT('Ctrl Pts',(20.8835778142264,-17.3578962203056,
-13.5233907858459));
#121132=CARTESIAN_POINT('Ctrl Pts',(21.2379147072037,-19.8965966223211,
-13.6505665925274));
#121133=CARTESIAN_POINT('Ctrl Pts',(19.2950652667951,-21.5686882516355,
-13.7777423992088));
#121134=CARTESIAN_POINT('Ctrl Pts',(16.8374732677398,-20.8401308200636,
-13.9049182058902));
#121135=CARTESIAN_POINT('Ctrl Pts',(16.1198268338089,-18.3793305516987,
-14.0320940125717));
#121136=CARTESIAN_POINT('Ctrl Pts',(17.8005220259727,-16.4439189582757,
-14.1592698192531));
#121137=CARTESIAN_POINT('Ctrl Pts',(20.3376253211293,-16.809516051569,-14.2864456259346));
#121138=CARTESIAN_POINT('Ctrl Pts',(21.4035019163622,-19.140709189997,-14.413621432616));
#121139=CARTESIAN_POINT('Ctrl Pts',(20.0202761913079,-21.2987733592159,
-14.5407972392974));
#121140=CARTESIAN_POINT('Ctrl Pts',(17.4569718960327,-21.303818628536,-14.6679730459788));
#121141=CARTESIAN_POINT('Ctrl Pts',(16.0652616248443,-19.1512162765007,
-14.7951488526603));
#121142=CARTESIAN_POINT('Ctrl Pts',(17.1219531722769,-16.8158453555327,
-14.9223246593417));
#121143=CARTESIAN_POINT('Ctrl Pts',(19.6575976292351,-16.4402637361534,
-15.0495004660232));
#121144=CARTESIAN_POINT('Ctrl Pts',(21.3458985863041,-18.369044242919,-15.1766762727046));
#121145=CARTESIAN_POINT('Ctrl Pts',(20.6379447031482,-20.8326504744915,
-15.303852079386));
#121146=CARTESIAN_POINT('Ctrl Pts',(18.1832397269893,-21.5708766220509,
-15.4310278860674));
#121147=CARTESIAN_POINT('Ctrl Pts',(16.2338231172801,-19.9064460146934,
-15.5582036927489));
#121148=CARTESIAN_POINT('Ctrl Pts',(16.578163618988,-17.3663704284554,-15.6853794994303));
#121149=CARTESIAN_POINT('Ctrl Pts',(18.9003501939781,-16.2810115588392,
-15.8125553061118));
#121150=CARTESIAN_POINT('Ctrl Pts',(21.0699207908507,-17.6461188037487,
-15.9397311127932));
#121151=CARTESIAN_POINT('Ctrl Pts',(21.0964290457131,-20.2092909940909,
-16.0669069194746));
#121152=CARTESIAN_POINT('Ctrl Pts',(18.955555280017,-21.6189767336345,-16.194082726156));
#121153=CARTESIAN_POINT('Ctrl Pts',(16.6114182961767,-20.5818768513131,
-16.3212585328375));
#121154=CARTESIAN_POINT('Ctrl Pts',(16.214618283316,-18.0494661194781,-16.4484343395189));
#121155=CARTESIAN_POINT('Ctrl Pts',(18.1291946250482,-16.3450742054518,
-16.5756101462004));
#121156=CARTESIAN_POINT('Ctrl Pts',(20.5986423598435,-17.0323749038605,
-16.7027859528818));
#121157=CARTESIAN_POINT('Ctrl Pts',(21.3573964622394,-19.4808124826067,
-16.8299617595632));
#121158=CARTESIAN_POINT('Ctrl Pts',(19.7093471368785,-21.4440974303655,
-16.9571375662447));
#121159=CARTESIAN_POINT('Ctrl Pts',(17.1664773503022,-21.1210376627748,
-17.0843133729261));
#121160=CARTESIAN_POINT('Ctrl Pts',(16.0617123033954,-18.8080204652485,
-17.2114891796075));
#121161=CARTESIAN_POINT('Ctrl Pts',(17.4086053572432,-16.6270955544791,
-17.338664986289));
#121162=CARTESIAN_POINT('Ctrl Pts',(19.9714657325515,-16.579126172631,-17.4658407929704));
#121163=CARTESIAN_POINT('Ctrl Pts',(21.3990281040287,-18.708121250235,-17.5930165996518));
#121164=CARTESIAN_POINT('Ctrl Pts',(20.3815926003592,-21.0608599439249,
-17.7201924063333));
#121165=CARTESIAN_POINT('Ctrl Pts',(17.8525931469884,-21.4788505296758,
-17.8473682130147));
#121166=CARTESIAN_POINT('Ctrl Pts',(16.1322297749793,-19.5786125884764,
-17.9745440196961));
#121167=CARTESIAN_POINT('Ctrl Pts',(16.7988291003494,-17.1034964893213,
-18.1017198263776));
#121168=CARTESIAN_POINT('Ctrl Pts',(19.2408276159067,-16.3242676301314,
-18.228895633059));
#121169=CARTESIAN_POINT('Ctrl Pts',(21.2178432511203,-17.955820124861,-18.3560714397405));
#121170=CARTESIAN_POINT('Ctrl Pts',(20.9160868681659,-20.5013058250774,
-18.4832472464219));
#121171=CARTESIAN_POINT('Ctrl Pts',(18.6124012191849,-21.6253995916595,
-18.6104230531033));
#121172=CARTESIAN_POINT('Ctrl Pts',(16.4202749044646,-20.2968151625747,
-18.7375988597848));
#121173=CARTESIAN_POINT('Ctrl Pts',(16.3508477586638,-17.7344462908773,
-18.8647746664662));
#121174=CARTESIAN_POINT('Ctrl Pts',(18.4678148796782,-16.2891073766096,
-18.9919504731476));
#121175=CARTESIAN_POINT('Ctrl Pts',(20.8289903263147,-17.286807168058,-19.119126279829));
#121176=CARTESIAN_POINT('Ctrl Pts',(21.2681421801737,-19.8122180263779,
-19.2463020865105));
#121177=CARTESIAN_POINT('Ctrl Pts',(19.3823758667575,-21.5484322422587,
-19.3734778931919));
#121178=CARTESIAN_POINT('Ctrl Pts',(16.9017649452107,-20.9025810178173,
-19.5006536998734));
#121179=CARTESIAN_POINT('Ctrl Pts',(16.1021159518554,-18.4671927970664,
-19.6278295065548));
#121180=CARTESIAN_POINT('Ctrl Pts',(17.7170572450437,-16.4765850543542,
-19.7550053132362));
#121181=CARTESIAN_POINT('Ctrl Pts',(20.2649803481551,-16.757016959998,-19.8821811199177));
#121182=CARTESIAN_POINT('Ctrl Pts',(21.4083240999114,-19.0512094198929,
-20.0093569265991));
#121183=CARTESIAN_POINT('Ctrl Pts',(20.0981412947811,-21.2543836816181,
-20.1365327332805));
#121184=CARTESIAN_POINT('Ctrl Pts',(17.5364438714413,-21.345263264656,-20.2637085399619));
#121185=CARTESIAN_POINT('Ctrl Pts',(16.0734291899427,-19.2404734101847,
-20.3908843466434));
#121186=CARTESIAN_POINT('Ctrl Pts',(17.0513243981187,-16.8710250544057,
-20.5180601533248));
#121187=CARTESIAN_POINT('Ctrl Pts',(19.5729675179493,-16.4107460050722,
-20.6452359600063));
#121188=CARTESIAN_POINT('Ctrl Pts',(21.3249148566822,-18.2819021506609,
-20.7724117666877));
#121189=CARTESIAN_POINT('Ctrl Pts',(20.6998492912724,-20.7678461580482,
-20.8995875733692));
#121190=CARTESIAN_POINT('Ctrl Pts',(18.2712569976611,-21.5878357442275,
-21.0267633800505));
#121191=CARTESIAN_POINT('Ctrl Pts',(16.2671680424845,-19.989664109829,-21.153939186732));
#121192=CARTESIAN_POINT('Ctrl Pts',(16.5263110482178,-17.4393951028376,
-21.2811149934134));
#121193=CARTESIAN_POINT('Ctrl Pts',(18.8107430407941,-16.2770494228818,
-21.4082908000949));
#121194=CARTESIAN_POINT('Ctrl Pts',(21.0250158365398,-17.568415239189,-21.5354666067763));
#121195=CARTESIAN_POINT('Ctrl Pts',(21.1369463139771,-20.1298851974028,
-21.6626424134577));
#121196=CARTESIAN_POINT('Ctrl Pts',(19.0452436034431,-21.6092686761098,
-21.7898182201392));
#121197=CARTESIAN_POINT('Ctrl Pts',(16.6662107583285,-20.6535950540795,
-21.9169940268206));
#121198=CARTESIAN_POINT('Ctrl Pts',(16.1877691759169,-18.1311075337387,
-22.044169833502));
#121199=CARTESIAN_POINT('Ctrl Pts',(17.4210581833076,-16.960478579468,-22.128953704623));
#121200=CARTESIAN_POINT('Ctrl Pts',(18.1489775593156,-16.7656980002009,
-22.1713456401835));
#121201=CARTESIAN_POINT('Ctrl Pts',(20.5799312301559,-17.397553415447,0.171094886838164));
#121202=CARTESIAN_POINT('Ctrl Pts',(21.0977302932135,-18.0124050913494,
0.128684295257136));
#121203=CARTESIAN_POINT('Ctrl Pts',(21.4611752643293,-19.7893203209783,
0.0438817681156306));
#121204=CARTESIAN_POINT('Ctrl Pts',(19.5021063818899,-21.7021724412225,
-0.083312694586353));
#121205=CARTESIAN_POINT('Ctrl Pts',(16.8390406066394,-21.0844924660501,
-0.210488501267787));
#121206=CARTESIAN_POINT('Ctrl Pts',(15.9143177655174,-18.5139387940262,
-0.337664307949222));
#121207=CARTESIAN_POINT('Ctrl Pts',(17.5765589760555,-16.343449345859,-0.464840114630656));
#121208=CARTESIAN_POINT('Ctrl Pts',(20.3006391625102,-16.567091249899,-0.592015921312091));
#121209=CARTESIAN_POINT('Ctrl Pts',(21.5874465485414,-18.9782470197745,
-0.719191727993525));
#121210=CARTESIAN_POINT('Ctrl Pts',(20.2563827322944,-21.3655780685178,
-0.84636753467496));
#121211=CARTESIAN_POINT('Ctrl Pts',(17.5286330090264,-21.5384685392327,
-0.973543341356393));
#121212=CARTESIAN_POINT('Ctrl Pts',(15.906729696796,-19.3385034339308,-1.10071914803782));
#121213=CARTESIAN_POINT('Ctrl Pts',(16.8786729593171,-16.7839097205383,
-1.22789495471926));
#121214=CARTESIAN_POINT('Ctrl Pts',(19.5527628216649,-16.2184227996018,
-1.35507076140069));
#121215=CARTESIAN_POINT('Ctrl Pts',(21.4756890313297,-18.1608136783876,
-1.48224656808212));
#121216=CARTESIAN_POINT('Ctrl Pts',(20.8832855061817,-20.8290738921377,
-1.60942237476356));
#121217=CARTESIAN_POINT('Ctrl Pts',(18.3190460414365,-21.7752327234411,
-1.73659818144499));
#121218=CARTESIAN_POINT('Ctrl Pts',(16.1355010202711,-20.1312521052755,
-1.86377398812643));
#121219=CARTESIAN_POINT('Ctrl Pts',(16.3359175623115,-17.4053801752063,
-1.99094979480786));
#121220=CARTESIAN_POINT('Ctrl Pts',(18.7364258834009,-16.0984363025981,
-2.1181256014893));
#121221=CARTESIAN_POINT('Ctrl Pts',(21.134708615211,-17.4094598221888,-2.24530140817073));
#121222=CARTESIAN_POINT('Ctrl Pts',(21.3304901931037,-20.135668311675,-2.37247721485217));
#121223=CARTESIAN_POINT('Ctrl Pts',(19.1441531773822,-21.7759345412849,
-2.4996530215336));
#121224=CARTESIAN_POINT('Ctrl Pts',(16.5815260772467,-20.8254161287028,
-2.62682882821504));
#121225=CARTESIAN_POINT('Ctrl Pts',(15.9936602042319,-18.1561546817078,
-2.75400463489647));
#121226=CARTESIAN_POINT('Ctrl Pts',(17.9198860088567,-16.2170319255978,
-2.8811804415779));
#121227=CARTESIAN_POINT('Ctrl Pts',(20.5930108709022,-16.7870726228123,
-3.00835624825934));
#121228=CARTESIAN_POINT('Ctrl Pts',(21.5606086420394,-19.3432998199575,
-3.13553205494077));
#121229=CARTESIAN_POINT('Ctrl Pts',(19.9349684232667,-21.5405337181072,
-3.26270786162221));
#121230=CARTESIAN_POINT('Ctrl Pts',(17.2075142166313,-21.3629485929295,
-3.38988366830364));
#121231=CARTESIAN_POINT('Ctrl Pts',(15.8805159718553,-18.9734677738181,
-3.51705947498508));
#121232=CARTESIAN_POINT('Ctrl Pts',(17.1714122157033,-16.5642916048074,
-3.64423528166651));
#121233=CARTESIAN_POINT('Ctrl Pts',(19.8958857665108,-16.3456896904175,
-3.77141108834795));
#121234=CARTESIAN_POINT('Ctrl Pts',(21.5544012413067,-18.5182157192451,
-3.89858689502938));
#121235=CARTESIAN_POINT('Ctrl Pts',(20.6253736310478,-21.0887119019572,
-4.02576270171081));
#121236=CARTESIAN_POINT('Ctrl Pts',(17.9611281061891,-21.6989075339308,
-4.15293850839225));
#121237=CARTESIAN_POINT('Ctrl Pts',(16.0059445740623,-19.7889859958273,
-4.28011431507368));
#121238=CARTESIAN_POINT('Ctrl Pts',(16.5535825730174,-17.1111817557645,
-4.40729012175512));
#121239=CARTESIAN_POINT('Ctrl Pts',(19.101618229261,-16.1222140007207,-4.53446592843655));
#121240=CARTESIAN_POINT('Ctrl Pts',(21.3123869771181,-17.7293992636892,
-4.66164173511799));
#121241=CARTESIAN_POINT('Ctrl Pts',(21.1576457062134,-20.4582448190627,
-4.78881754179942));
#121242=CARTESIAN_POINT('Ctrl Pts',(18.7793599282756,-21.8052042410432,
-4.91599334848085));
#121243=CARTESIAN_POINT('Ctrl Pts',(16.3594592314994,-20.5345258616938,
-5.04316915516229));
#121244=CARTESIAN_POINT('Ctrl Pts',(16.1180523092011,-17.8119782268727,
-5.17034496184372));
#121245=CARTESIAN_POINT('Ctrl Pts',(18.2766150291857,-16.1353298111647,
-5.29752076852516));
#121246=CARTESIAN_POINT('Ctrl Pts',(20.8548000713794,-17.0428014714449,
-5.42469657520659));
#121247=CARTESIAN_POINT('Ctrl Pts',(21.4872826797803,-19.7018442834496,
-5.55187238188803));
#121248=CARTESIAN_POINT('Ctrl Pts',(19.5937993174784,-21.6729515059744,
-5.67904818856947));
#121249=CARTESIAN_POINT('Ctrl Pts',(16.9115034465541,-21.1477546030643,
-5.80622399525089));
#121250=CARTESIAN_POINT('Ctrl Pts',(15.901235046523,-18.6080891357435,-5.93339980193234));
#121251=CARTESIAN_POINT('Ctrl Pts',(17.4898526700851,-16.3839405408623,
-6.06057560861376));
#121252=CARTESIAN_POINT('Ctrl Pts',(20.2198982483519,-16.515827107994,-6.1877514152952));
#121253=CARTESIAN_POINT('Ctrl Pts',(21.5867244090021,-18.8827510975986,
-6.31492722197664));
#121254=CARTESIAN_POINT('Ctrl Pts',(20.3363529844383,-21.3132066570849,
-6.44210302865807));
#121255=CARTESIAN_POINT('Ctrl Pts',(17.6159221498948,-21.577401661709,-6.5692788353395));
#121256=CARTESIAN_POINT('Ctrl Pts',(15.921258347085,-19.4329535925197,-6.69645464202094));
#121257=CARTESIAN_POINT('Ctrl Pts',(16.8071104323889,-16.8472604535401,
-6.82363044870237));
#121258=CARTESIAN_POINT('Ctrl Pts',(19.4607640997214,-16.1925352135684,
-6.95080625538382));
#121259=CARTESIAN_POINT('Ctrl Pts',(21.4476568136269,-18.0694476434471,
-7.07798206206524));
#121260=CARTESIAN_POINT('Ctrl Pts',(20.9449378295665,-20.7560470830862,
-7.20515786874667));
#121261=CARTESIAN_POINT('Ctrl Pts',(18.4138206131569,-21.7875452957837,
-7.33233367542811));
#121262=CARTESIAN_POINT('Ctrl Pts',(16.1764481116018,-20.2176066933892,
-7.45950948210954));
#121263=CARTESIAN_POINT('Ctrl Pts',(16.2854707280793,-17.4865525022204,
-7.58668528879099));
#121264=CARTESIAN_POINT('Ctrl Pts',(18.6408669786781,-16.0999554343348,
-7.7138610954724));
#121265=CARTESIAN_POINT('Ctrl Pts',(21.0817069958525,-17.3299322375973,
-7.84103690215386));
#121266=CARTESIAN_POINT('Ctrl Pts',(21.3686715594619,-20.0480555359847,
-7.96821270883527));
#121267=CARTESIAN_POINT('Ctrl Pts',(19.2384884934243,-21.7606159089848,
-8.09538851551672));
#121268=CARTESIAN_POINT('Ctrl Pts',(16.6454685467572,-20.8964455078546,
-8.22256432219814));
#121269=CARTESIAN_POINT('Ctrl Pts',(15.9685465795588,-18.2483670391668,
-8.3497401288796));
#121270=CARTESIAN_POINT('Ctrl Pts',(17.8287564822182,-16.2458281396566,
-8.47691593556101));
#121271=CARTESIAN_POINT('Ctrl Pts',(20.5194711266931,-16.726033958043,-8.60409174224245));
#121272=CARTESIAN_POINT('Ctrl Pts',(21.5721268312631,-19.248425460891,-8.7312675489239));
#121273=CARTESIAN_POINT('Ctrl Pts',(20.0209773221669,-21.4988650016106,
-8.85844335560532));
#121274=CARTESIAN_POINT('Ctrl Pts',(17.2891059988037,-21.412713979622,-8.98561916228675));
#121275=CARTESIAN_POINT('Ctrl Pts',(15.8828352413023,-19.0690106104646,
-9.11279496896819));
#121276=CARTESIAN_POINT('Ctrl Pts',(17.0923311866634,-16.6179572687033,
-9.23997077564962));
#121277=CARTESIAN_POINT('Ctrl Pts',(19.8079563748028,-16.308243265877,-9.36714658233106));
#121278=CARTESIAN_POINT('Ctrl Pts',(21.5382932463106,-18.4240119765596,
-9.49432238901249));
#121279=CARTESIAN_POINT('Ctrl Pts',(20.6958651183971,-21.0241769281162,
-9.62149819569393));
#121280=CARTESIAN_POINT('Ctrl Pts',(18.0535475114361,-21.7232481619313,
-9.74867400237536));
#121281=CARTESIAN_POINT('Ctrl Pts',(16.0355028290879,-19.8798712102337,
-9.87584980905679));
#121282=CARTESIAN_POINT('Ctrl Pts',(16.4931618134281,-17.1852300133289,
-10.0030256157383));
#121283=CARTESIAN_POINT('Ctrl Pts',(19.0066507518444,-16.1114906210823,
-10.1302014224197));
#121284=CARTESIAN_POINT('Ctrl Pts',(21.2699995480578,-17.6437422820975,
-10.2573772291012));
#121285=CARTESIAN_POINT('Ctrl Pts',(21.2067261608115,-20.3762391996566,
-10.3845530357826));
#121286=CARTESIAN_POINT('Ctrl Pts',(18.874879995715,-21.802085049785,-10.511728842464));
#121287=CARTESIAN_POINT('Ctrl Pts',(16.4137851785486,-20.613154762964,-10.6389046491454));
#121288=CARTESIAN_POINT('Ctrl Pts',(16.0813434512909,-17.9002180840159,
-10.7660804558269));
#121289=CARTESIAN_POINT('Ctrl Pts',(18.1825494650401,-16.1522260320353,
-10.8932562625082));
#121290=CARTESIAN_POINT('Ctrl Pts',(20.7896771177347,-16.9728528220917,
-11.0204320691897));
#121291=CARTESIAN_POINT('Ctrl Pts',(21.5108486046191,-19.6092243081515,
-11.1476078758711));
#121292=CARTESIAN_POINT('Ctrl Pts',(19.6844338474273,-21.6426332834231,
-11.2747836825526));
#121293=CARTESIAN_POINT('Ctrl Pts',(16.9860550257985,-21.2075532206898,
-11.4019594892341));
#121294=CARTESIAN_POINT('Ctrl Pts',(15.8913072282989,-18.7031430733949,
-11.5291352959155));
#121295=CARTESIAN_POINT('Ctrl Pts',(17.4045536114233,-16.4270437104573,
-11.6563111025968));
#121296=CARTESIAN_POINT('Ctrl Pts',(20.1374845413179,-16.4674350267135,
-11.7834869092783));
#121297=CARTESIAN_POINT('Ctrl Pts',(21.5828055146281,-18.7872604964662,
-11.9106627159598));
#121298=CARTESIAN_POINT('Ctrl Pts',(20.4145242450785,-21.2582242358244,
-12.0378385226412));
#121299=CARTESIAN_POINT('Ctrl Pts',(17.7044662857673,-21.613370379233,-12.1650143293227));
#121300=CARTESIAN_POINT('Ctrl Pts',(15.9389416091958,-19.5268743829703,
-12.2921901360041));
#121301=CARTESIAN_POINT('Ctrl Pts',(16.7377095252982,-16.9129668210605,
-12.4193659426856));
#121302=CARTESIAN_POINT('Ctrl Pts',(19.3679500481791,-16.1697456441557,
-12.5465417493669));
#121303=CARTESIAN_POINT('Ctrl Pts',(21.416580749233,-17.9790701525573,-12.6737175560484));
#121304=CARTESIAN_POINT('Ctrl Pts',(21.0041101126047,-20.6809974091509,
-12.8008933627298));
#121305=CARTESIAN_POINT('Ctrl Pts',(18.5089543465855,-21.7966768565304,
-12.9280691694113));
#121306=CARTESIAN_POINT('Ctrl Pts',(16.2202639996657,-20.3025418486013,
-13.0552449760926));
#121307=CARTESIAN_POINT('Ctrl Pts',(16.2377704130005,-17.5693685186612,
-13.1824207827741));
#121308=CARTESIAN_POINT('Ctrl Pts',(18.545412538926,-16.1046737570615,-13.3095965894556));
#121309=CARTESIAN_POINT('Ctrl Pts',(21.0260719553289,-17.2522240983603,
-13.436772396137));
#121310=CARTESIAN_POINT('Ctrl Pts',(21.4038976147472,-19.9592133294229,
-13.5639482028184));
#121311=CARTESIAN_POINT('Ctrl Pts',(19.3322579251698,-21.7421468454496,
-13.6911240094999));
#121312=CARTESIAN_POINT('Ctrl Pts',(16.7117537213236,-20.96529380682,-13.8182998161813));
#121313=CARTESIAN_POINT('Ctrl Pts',(15.9465349634034,-18.3413686595396,
-13.9454756228628));
#121314=CARTESIAN_POINT('Ctrl Pts',(17.7386423669686,-16.2776598670762,
-14.0726514295442));
#121315=CARTESIAN_POINT('Ctrl Pts',(20.443928619978,-16.6674921583018,-14.1998272362256));
#121316=CARTESIAN_POINT('Ctrl Pts',(21.5804614942969,-19.1532186017375,
-14.3270030429069));
#121317=CARTESIAN_POINT('Ctrl Pts',(20.1055426189236,-21.454339467114,-14.4541788495885));
#121318=CARTESIAN_POINT('Ctrl Pts',(17.3723185182233,-21.4597191841168,
-14.5813546562699));
#121319=CARTESIAN_POINT('Ctrl Pts',(15.8883526615688,-19.1644221962985,
-14.7085304629514));
#121320=CARTESIAN_POINT('Ctrl Pts',(17.0150916171319,-16.6742410277849,
-14.8357062696328));
#121321=CARTESIAN_POINT('Ctrl Pts',(19.7188223264901,-16.2737623426128,
-14.9628820763142));
#121322=CARTESIAN_POINT('Ctrl Pts',(21.5190396762608,-18.3304004779172,
-15.0900578829957));
#121323=CARTESIAN_POINT('Ctrl Pts',(20.7641559821193,-20.9573175939151,
-15.2172336896771));
#121324=CARTESIAN_POINT('Ctrl Pts',(18.1467301800744,-21.7444802815428,
-15.3444094963585));
#121325=CARTESIAN_POINT('Ctrl Pts',(16.0680879877353,-19.9697156317281,
-15.4715853030399));
#121326=CARTESIAN_POINT('Ctrl Pts',(16.4352546014886,-17.2612600563589,
-15.5987611097214));
#121327=CARTESIAN_POINT('Ctrl Pts',(18.9113774421457,-16.1039534401246,
-15.7259369164028));
#121328=CARTESIAN_POINT('Ctrl Pts',(21.2247674889198,-17.5595527728704,
-15.8531127230842));
#121329=CARTESIAN_POINT('Ctrl Pts',(21.2530329590753,-20.2926360114859,
-15.9802885297657));
#121330=CARTESIAN_POINT('Ctrl Pts',(18.9702420380974,-21.7957689188181,
-16.1074643364471));
#121331=CARTESIAN_POINT('Ctrl Pts',(16.4707137099997,-20.6899203473398,
-16.2346401431286));
#121332=CARTESIAN_POINT('Ctrl Pts',(16.0476100775874,-17.9896377246791,
-16.3618159498099));
#121333=CARTESIAN_POINT('Ctrl Pts',(18.0891024628257,-16.1722627586861,
-16.4889917564913));
#121334=CARTESIAN_POINT('Ctrl Pts',(20.722248311566,-16.9051241816477,-16.6161675631729));
#121335=CARTESIAN_POINT('Ctrl Pts',(21.5312997390521,-19.5158671245064,
-16.7433433698543));
#121336=CARTESIAN_POINT('Ctrl Pts',(19.7740022759604,-21.6092969781711,
-16.8705191765357));
#121337=CARTESIAN_POINT('Ctrl Pts',(17.062567274496,-21.2648217848151,-16.9976949832172));
#121338=CARTESIAN_POINT('Ctrl Pts',(15.8845680578669,-18.7984761538005,
-17.1248707898986));
#121339=CARTESIAN_POINT('Ctrl Pts',(17.3207457924526,-16.4729791229096,
-17.2520465965799));
#121340=CARTESIAN_POINT('Ctrl Pts',(20.0534965460147,-16.4218298813604,
-17.3792224032615));
#121341=CARTESIAN_POINT('Ctrl Pts',(21.5756911157996,-18.6919546835953,
-17.5063982099429));
#121342=CARTESIAN_POINT('Ctrl Pts',(20.4908104620813,-21.2006549233977,
-17.6335740166242));
#121343=CARTESIAN_POINT('Ctrl Pts',(17.7941652493564,-21.6463538382498,
-17.7607498233058));
#121344=CARTESIAN_POINT('Ctrl Pts',(15.9597600876265,-19.6201503369626,
-17.8879256299872));
#121345=CARTESIAN_POINT('Ctrl Pts',(16.6705478567457,-16.9809603716076,
-18.0151014366687));
#121346=CARTESIAN_POINT('Ctrl Pts',(19.274424895027,-16.1500769287699,-18.1422772433501));
#121347=CARTESIAN_POINT('Ctrl Pts',(21.382495634653,-17.8897839968585,-18.2694530500315));
#121348=CARTESIAN_POINT('Ctrl Pts',(21.0607360137014,-20.6040083192082,
-18.3966288567128));
#121349=CARTESIAN_POINT('Ctrl Pts',(18.6043405136283,-21.8026175440015,
-18.5238046633944));
#121350=CARTESIAN_POINT('Ctrl Pts',(16.2668995448691,-20.3859621012267,
-18.6509804700757));
#121351=CARTESIAN_POINT('Ctrl Pts',(16.1928701178928,-17.6537354327361,
-18.7781562767572));
#121352=CARTESIAN_POINT('Ctrl Pts',(18.4501696379737,-16.1125859244869,
-18.9053320834387));
#121353=CARTESIAN_POINT('Ctrl Pts',(20.9678658976898,-17.1764225982197,
-19.0325078901201));
#121354=CARTESIAN_POINT('Ctrl Pts',(21.4361288476046,-19.8692413302184,
-19.1596836968014));
#121355=CARTESIAN_POINT('Ctrl Pts',(19.4253562890682,-21.7205480781417,
-19.286859503483));
#121356=CARTESIAN_POINT('Ctrl Pts',(16.7803072530527,-21.0318837883171,
-19.4140353101644));
#121357=CARTESIAN_POINT('Ctrl Pts',(15.9276500383911,-18.4350552370649,
-19.5412111168458));
#121358=CARTESIAN_POINT('Ctrl Pts',(17.6496447589923,-16.3124913778111,
-19.6683869235273));
#121359=CARTESIAN_POINT('Ctrl Pts',(20.366468058119,-16.6115129354638,-19.7955627302086));
#121360=CARTESIAN_POINT('Ctrl Pts',(21.5856033373152,-19.0577859490064,
-19.9227385368901));
#121361=CARTESIAN_POINT('Ctrl Pts',(20.1885693504001,-21.4070072261248,
-20.0499143435716));
#121362=CARTESIAN_POINT('Ctrl Pts',(17.45705864015,-21.5039111587085,-20.1770901502529));
#121363=CARTESIAN_POINT('Ctrl Pts',(15.8970616493438,-19.2595961283962,
-20.3042659569345));
#121364=CARTESIAN_POINT('Ctrl Pts',(16.9397809066213,-16.7330785536716,
-20.4314417636159));
#121365=CARTESIAN_POINT('Ctrl Pts',(19.6285821391516,-16.2422878999811,
-20.5586175702973));
#121366=CARTESIAN_POINT('Ctrl Pts',(21.4966649485975,-18.2374817919912,
-20.6857933769788));
#121367=CARTESIAN_POINT('Ctrl Pts',(20.8301641858729,-20.8882174407032,
-20.8129691836602));
#121368=CARTESIAN_POINT('Ctrl Pts',(18.2405820594323,-21.7625636131024,
-20.9401449903416));
#121369=CARTESIAN_POINT('Ctrl Pts',(16.1036433267455,-20.0584502012673,
-21.0673207970231));
#121370=CARTESIAN_POINT('Ctrl Pts',(16.3799647569026,-17.3391254897899,
-21.1944966037045));
#121371=CARTESIAN_POINT('Ctrl Pts',(18.8158302879787,-16.0997286567039,
-21.3216724103859));
#121372=CARTESIAN_POINT('Ctrl Pts',(21.1768858138531,-17.4766982886188,
-21.4488482170674));
#121373=CARTESIAN_POINT('Ctrl Pts',(21.2962360911878,-20.207966455225,-21.5760240237488));
#121374=CARTESIAN_POINT('Ctrl Pts',(19.0658757432302,-21.7854173203574,
-21.7031998304301));
#121375=CARTESIAN_POINT('Ctrl Pts',(16.5291383294904,-20.7663927039858,
-21.8303756371117));
#121376=CARTESIAN_POINT('Ctrl Pts',(16.0189811599981,-18.0766910961744,
-21.9575514437931));
#121377=CARTESIAN_POINT('Ctrl Pts',(17.3340241084075,-16.8284618958069,
-22.0423353149141));
#121378=CARTESIAN_POINT('Ctrl Pts',(18.110196795177,-16.6207694362802,-22.0847272504745));
#121379=CARTESIAN_POINT('Ctrl Pts',(20.694689575575,-17.3009161652768,0.2577132765471));
#121380=CARTESIAN_POINT('Ctrl Pts',(21.2446793089921,-17.9539921042784,
0.215302684966073));
#121381=CARTESIAN_POINT('Ctrl Pts',(21.6307190240803,-19.8413750741844,
0.130500157824568));
#121382=CARTESIAN_POINT('Ctrl Pts',(19.5498582244566,-21.8731458956047,
0.00330569512258449));
#121383=CARTESIAN_POINT('Ctrl Pts',(16.721234265284,-21.2170658268692,-0.123870111558849));
#121384=CARTESIAN_POINT('Ctrl Pts',(15.7390230077546,-18.486705288049,-0.251045918240284));
#121385=CARTESIAN_POINT('Ctrl Pts',(17.504602873543,-16.1812802725366,-0.378221724921718));
#121386=CARTESIAN_POINT('Ctrl Pts',(20.3980344041213,-16.4188256061598,
-0.505397531603153));
#121387=CARTESIAN_POINT('Ctrl Pts',(21.7648403751927,-18.9798787515055,
-0.632573338284587));
#121388=CARTESIAN_POINT('Ctrl Pts',(20.3510266283393,-21.5156260340964,
-0.759749144966022));
#121389=CARTESIAN_POINT('Ctrl Pts',(17.4536974322035,-21.6992648057414,
-0.886924951647455));
#121390=CARTESIAN_POINT('Ctrl Pts',(15.7309632019515,-19.3625316825741,
-1.01410075832889));
#121391=CARTESIAN_POINT('Ctrl Pts',(16.7633304926413,-16.6491233053535,
-1.14127656501032));
#121392=CARTESIAN_POINT('Ctrl Pts',(19.6036638873005,-16.0484810425805,
-1.26845237169176));
#121393=CARTESIAN_POINT('Ctrl Pts',(21.6461350868215,-18.1116269959678,
-1.39562817837319));
#121394=CARTESIAN_POINT('Ctrl Pts',(21.016902861202,-20.9457683228794,-1.52280398505463));
#121395=CARTESIAN_POINT('Ctrl Pts',(18.2932490729839,-21.9507482089492,
-1.64997979173606));
#121396=CARTESIAN_POINT('Ctrl Pts',(15.9739568421265,-20.2045641649137,
-1.7771555984175));
#121397=CARTESIAN_POINT('Ctrl Pts',(16.1868329332462,-17.3092295011259,
-1.90433140509893));
#121398=CARTESIAN_POINT('Ctrl Pts',(18.7365766963677,-15.9210351930051,
-2.03150721178036));
#121399=CARTESIAN_POINT('Ctrl Pts',(21.2839565091815,-17.3135627726908,
-2.1586830184618));
#121400=CARTESIAN_POINT('Ctrl Pts',(21.4919094884653,-20.2092549192115,
-2.28585882514323));
#121401=CARTESIAN_POINT('Ctrl Pts',(19.1696516895889,-21.951493657592,-2.41303463182467));
#121402=CARTESIAN_POINT('Ctrl Pts',(16.447710503894,-20.9418831626308,-2.5402104385061));
#121403=CARTESIAN_POINT('Ctrl Pts',(15.8232980283766,-18.1066783575389,
-2.66738624518754));
#121404=CARTESIAN_POINT('Ctrl Pts',(17.8692739529578,-16.0470037003502,
-2.79456205186897));
#121405=CARTESIAN_POINT('Ctrl Pts',(20.7085823549184,-16.6524828397803,
-2.9217378585504));
#121406=CARTESIAN_POINT('Ctrl Pts',(21.7363340025561,-19.3676262516076,
-3.04891366523184));
#121407=CARTESIAN_POINT('Ctrl Pts',(20.0096305487582,-21.7014583732073,
-3.17608947191327));
#121408=CARTESIAN_POINT('Ctrl Pts',(17.1126152410121,-21.5128330885679,
-3.30326527859471));
#121409=CARTESIAN_POINT('Ctrl Pts',(15.703119815162,-18.9748023881108,-3.43044108527614));
#121410=CARTESIAN_POINT('Ctrl Pts',(17.0742688412544,-16.4158519119851,
-3.55761689195758));
#121411=CARTESIAN_POINT('Ctrl Pts',(19.9681181909656,-16.1836598954335,
-3.68479269863901));
#121412=CARTESIAN_POINT('Ctrl Pts',(21.7297406984776,-18.4912481022967,
-3.81196850532045));
#121413=CARTESIAN_POINT('Ctrl Pts',(20.7429570517748,-21.221547577794,-3.93914431200188));
#121414=CARTESIAN_POINT('Ctrl Pts',(17.9130800000052,-21.8696780146852,
-4.06632011868332));
#121415=CARTESIAN_POINT('Ctrl Pts',(15.8363460961894,-19.8410199646181,
-4.19349592536474));
#121416=CARTESIAN_POINT('Ctrl Pts',(16.4180298004353,-16.9967412758189,
-4.32067173204619));
#121417=CARTESIAN_POINT('Ctrl Pts',(19.1244724174598,-15.9462911094113,
-4.44784753872761));
#121418=CARTESIAN_POINT('Ctrl Pts',(21.4726808269163,-17.6533922947864,
-4.57502334540905));
#121419=CARTESIAN_POINT('Ctrl Pts',(21.3083195593796,-20.5518854490104,
-4.70219915209049));
#121420=CARTESIAN_POINT('Ctrl Pts',(18.7821798764038,-21.9825830038574,
-4.82937495877192));
#121421=CARTESIAN_POINT('Ctrl Pts',(16.2118381472079,-20.6329087518601,
-4.95655076545335));
#121422=CARTESIAN_POINT('Ctrl Pts',(15.9554233749293,-17.7411050489944,
-5.08372657213479));
#121423=CARTESIAN_POINT('Ctrl Pts',(18.2481801982382,-15.9602223070596,
-5.21090237881622));
#121424=CARTESIAN_POINT('Ctrl Pts',(20.9866465362858,-16.9241099077319,
-5.33807818549766));
#121425=CARTESIAN_POINT('Ctrl Pts',(21.6584494923035,-19.7484608030061,
-5.46525399217908));
#121426=CARTESIAN_POINT('Ctrl Pts',(19.6472515509388,-21.8421083454547,
-5.59242979886053));
#121427=CARTESIAN_POINT('Ctrl Pts',(16.7982019943716,-21.2842608613028,
-5.71960560554195));
#121428=CARTESIAN_POINT('Ctrl Pts',(15.7251269587939,-18.5867087933401,
-5.8467814122234));
#121429=CARTESIAN_POINT('Ctrl Pts',(17.4125061868001,-16.2242887349586,
-5.97395721890483));
#121430=CARTESIAN_POINT('Ctrl Pts',(20.3122739672608,-16.3643744613978,
-6.10113302558626));
#121431=CARTESIAN_POINT('Ctrl Pts',(21.7640733414898,-18.8784460133507,
-6.2283088322677));
#121432=CARTESIAN_POINT('Ctrl Pts',(20.4359684924635,-21.459998782779,-6.35548463894913));
#121433=CARTESIAN_POINT('Ctrl Pts',(17.54641318768,-21.7406183329676,-6.48266044563057));
#121434=CARTESIAN_POINT('Ctrl Pts',(15.7463950732497,-19.4628536438322,
-6.609836252312));
#121435=CARTESIAN_POINT('Ctrl Pts',(16.687319047438,-16.7164124436336,-6.73701205899344));
#121436=CARTESIAN_POINT('Ctrl Pts',(19.5059457642557,-16.0209840701888,
-6.86418786567487));
#121437=CARTESIAN_POINT('Ctrl Pts',(21.6163601547263,-18.0145808929804,
-6.99136367235631));
#121438=CARTESIAN_POINT('Ctrl Pts',(21.0823880026828,-20.8682015636709,
-7.11853947903774));
#121439=CARTESIAN_POINT('Ctrl Pts',(18.3939156155756,-21.9638262325755,
-7.24571528571917));
#121440=CARTESIAN_POINT('Ctrl Pts',(16.0174495431603,-20.2962872681105,
-7.37289109240061));
#121441=CARTESIAN_POINT('Ctrl Pts',(16.1332499067586,-17.3954481710316,
-7.50006689908204));
#121442=CARTESIAN_POINT('Ctrl Pts',(18.6350770601501,-15.9226487665292,
-7.62724270576348));
#121443=CARTESIAN_POINT('Ctrl Pts',(21.2276598710039,-17.2290910959936,
-7.75441851244491));
#121444=CARTESIAN_POINT('Ctrl Pts',(21.5324645241983,-20.1161954090971,
-7.88159431912634));
#121445=CARTESIAN_POINT('Ctrl Pts',(19.2698516687381,-21.9352226924704,
-8.00877012580778));
#121446=CARTESIAN_POINT('Ctrl Pts',(16.515628165916,-21.0173283151844,-8.13594593248921));
#121447=CARTESIAN_POINT('Ctrl Pts',(15.7966231331817,-18.204623397449,-8.26312173917066));
#121448=CARTESIAN_POINT('Ctrl Pts',(17.7724790615836,-16.0775901251306,
-8.39029754585207));
#121449=CARTESIAN_POINT('Ctrl Pts',(20.6304707722626,-16.5876495070077,
-8.51747335253352));
#121450=CARTESIAN_POINT('Ctrl Pts',(21.7485682576417,-19.2668537180634,
-8.64464915921495));
#121451=CARTESIAN_POINT('Ctrl Pts',(20.1009864718422,-21.6571991848217,
-8.77182496589638));
#121452=CARTESIAN_POINT('Ctrl Pts',(17.1992794428765,-21.5656923031035,
-8.89900077257782));
#121453=CARTESIAN_POINT('Ctrl Pts',(15.7055832695711,-19.0762849573276,
-9.02617657925925));
#121454=CARTESIAN_POINT('Ctrl Pts',(16.9902714816934,-16.4728538771981,
-9.15335238594069));
#121455=CARTESIAN_POINT('Ctrl Pts',(19.8747223813643,-16.1438854915773,
-9.28052819262213));
#121456=CARTESIAN_POINT('Ctrl Pts',(21.7126312973492,-18.3911878761916,
-9.40770399930354));
#121457=CARTESIAN_POINT('Ctrl Pts',(20.8178308727247,-21.1530005764741,
-9.53487980598501));
#121458=CARTESIAN_POINT('Ctrl Pts',(18.0112449595055,-21.8955318573441,
-9.66205561266641));
#121459=CARTESIAN_POINT('Ctrl Pts',(15.8677419367031,-19.9375553552922,
-9.78923141934787));
#121460=CARTESIAN_POINT('Ctrl Pts',(16.3538527869367,-17.0753929852239,
-9.91640722602929));
#121461=CARTESIAN_POINT('Ctrl Pts',(19.0236009765592,-15.9349010758452,
-10.0435830327107));
#121462=CARTESIAN_POINT('Ctrl Pts',(21.4276582448523,-17.5624101671002,
-10.1707588393921));
#121463=CARTESIAN_POINT('Ctrl Pts',(21.3604512607793,-20.4647816823687,
-10.2979346460736));
#121464=CARTESIAN_POINT('Ctrl Pts',(18.8836382608913,-21.9792698978844,
-10.4251104527551));
#121465=CARTESIAN_POINT('Ctrl Pts',(16.2695414442334,-20.7164258756515,
-10.5522862594364));
#121466=CARTESIAN_POINT('Ctrl Pts',(15.9164323909425,-17.8348306251289,
-10.6794620661178));
#121467=CARTESIAN_POINT('Ctrl Pts',(18.1482667409934,-15.9781689366991,
-10.8066378727993));
#121468=CARTESIAN_POINT('Ctrl Pts',(20.9174750014767,-16.8498126720757,
-10.9338136794807));
#121469=CARTESIAN_POINT('Ctrl Pts',(21.6834804698477,-19.6500828043623,
-11.0609894861622));
#121470=CARTESIAN_POINT('Ctrl Pts',(19.7435206725372,-21.8099052915517,
-11.1881652928436));
#121471=CARTESIAN_POINT('Ctrl Pts',(16.8773883160933,-21.3477770553498,
-11.315341099525));
#121472=CARTESIAN_POINT('Ctrl Pts',(15.7145819453165,-18.6876720695586,
-11.4425169062064));
#121473=CARTESIAN_POINT('Ctrl Pts',(17.321904233492,-16.2700715539058,-11.5696927128879));
#121474=CARTESIAN_POINT('Ctrl Pts',(20.2247367428907,-16.3129739282918,
-11.6968685195694));
#121475=CARTESIAN_POINT('Ctrl Pts',(21.7599108162444,-18.7770189270394,
-11.8240443262508));
#121476=CARTESIAN_POINT('Ctrl Pts',(20.5189995249,-21.401598199678,-11.9512201329322));
#121477=CARTESIAN_POINT('Ctrl Pts',(17.6404619590251,-21.7788231633232,
-12.0783959396136));
#121478=CARTESIAN_POINT('Ctrl Pts',(15.7651776731192,-19.5626133270521,
-12.2055717462951));
#121479=CARTESIAN_POINT('Ctrl Pts',(16.6136036062314,-16.7862036621481,
-12.3327475529765));
#121480=CARTESIAN_POINT('Ctrl Pts',(19.4073616239837,-15.9967777127422,
-12.4599233596579));
#121481=CARTESIAN_POINT('Ctrl Pts',(21.5833521452667,-17.9185847901141,
-12.5870991663394));
#121482=CARTESIAN_POINT('Ctrl Pts',(21.1452389240066,-20.7884861815747,
-12.7142749730208));
#121483=CARTESIAN_POINT('Ctrl Pts',(18.4949636483364,-21.973525486628,-12.8414507797022));
#121484=CARTESIAN_POINT('Ctrl Pts',(16.0639893890483,-20.3865026947222,
-12.9686265863837));
#121485=CARTESIAN_POINT('Ctrl Pts',(16.0825841457601,-17.4834127156872,
-13.0958023930651));
#121486=CARTESIAN_POINT('Ctrl Pts',(18.5336883833095,-15.9276604192025,
-13.2229781997465));
#121487=CARTESIAN_POINT('Ctrl Pts',(21.1685660964313,-17.1465519764151,
-13.350154006428));
#121488=CARTESIAN_POINT('Ctrl Pts',(21.5698805222909,-20.0218300365248,
-13.4773298131094));
#121489=CARTESIAN_POINT('Ctrl Pts',(19.3694505835445,-21.9156054392635,
-13.6045056197909));
#121490=CARTESIAN_POINT('Ctrl Pts',(16.5860341749072,-21.0904567935765,
-13.7316814264723));
#121491=CARTESIAN_POINT('Ctrl Pts',(15.773243092998,-18.3034067673804,-13.8588572331537));
#121492=CARTESIAN_POINT('Ctrl Pts',(17.6767627079645,-16.1114007758768,
-13.9860330398351));
#121493=CARTESIAN_POINT('Ctrl Pts',(20.5502319188267,-16.5254682650346,
-14.1132088465166));
#121494=CARTESIAN_POINT('Ctrl Pts',(21.7574210722316,-19.1657280134782,
-14.240384653198));
#121495=CARTESIAN_POINT('Ctrl Pts',(20.1908090465392,-21.6099055750122,
-14.3675604598796));
#121496=CARTESIAN_POINT('Ctrl Pts',(17.2876651404139,-21.6156197396974,
-14.4947362665609));
#121497=CARTESIAN_POINT('Ctrl Pts',(15.7114436982933,-19.1776281160963,
-14.6219120732423));
#121498=CARTESIAN_POINT('Ctrl Pts',(16.9082300619871,-16.5326367000369,
-14.7490878799237));
#121499=CARTESIAN_POINT('Ctrl Pts',(19.7800470237451,-16.1072609490722,
-14.8762636866052));
#121500=CARTESIAN_POINT('Ctrl Pts',(21.6921807662175,-18.2917567129154,
-15.0034394932866));
#121501=CARTESIAN_POINT('Ctrl Pts',(20.8903672610905,-21.0819847133387,
-15.130615299968));
#121502=CARTESIAN_POINT('Ctrl Pts',(18.1102206331594,-21.9180839410347,
-15.2577911066495));
#121503=CARTESIAN_POINT('Ctrl Pts',(15.9023528581907,-20.0329852487628,
-15.3849669133309));
#121504=CARTESIAN_POINT('Ctrl Pts',(16.2923455839892,-17.1561496842624,
-15.5121427200123));
#121505=CARTESIAN_POINT('Ctrl Pts',(18.9224046903134,-15.9268953214099,
-15.6393185266939));
#121506=CARTESIAN_POINT('Ctrl Pts',(21.3796141869889,-17.4729867419922,
-15.7664943333752));
#121507=CARTESIAN_POINT('Ctrl Pts',(21.4096368724374,-20.375981028881,-15.8936701400568));
#121508=CARTESIAN_POINT('Ctrl Pts',(18.9849287961779,-21.9725611040017,
-16.0208459467382));
#121509=CARTESIAN_POINT('Ctrl Pts',(16.3300091238228,-20.7979638433666,
-16.1480217534195));
#121510=CARTESIAN_POINT('Ctrl Pts',(15.8806018718589,-17.9298093298801,
-16.2751975601011));
#121511=CARTESIAN_POINT('Ctrl Pts',(18.0490103006032,-15.9994513119205,
-16.4023733667824));
#121512=CARTESIAN_POINT('Ctrl Pts',(20.8458542632885,-16.7778734594348,
-16.5295491734638));
#121513=CARTESIAN_POINT('Ctrl Pts',(21.7052030158649,-19.5509217664061,
-16.6567249801453));
#121514=CARTESIAN_POINT('Ctrl Pts',(19.8386574150423,-21.7744965259768,
-16.7839007868268));
#121515=CARTESIAN_POINT('Ctrl Pts',(16.9586571986901,-21.4086059068554,
-16.9110765935081));
#121516=CARTESIAN_POINT('Ctrl Pts',(15.7074238123383,-18.7889318423525,
-17.0382524001897));
#121517=CARTESIAN_POINT('Ctrl Pts',(17.2328862276622,-16.31886269134,-17.165428206871));
#121518=CARTESIAN_POINT('Ctrl Pts',(20.135527359478,-16.2645335900898,-17.2926040135526));
#121519=CARTESIAN_POINT('Ctrl Pts',(21.7523541275707,-18.6757881169556,
-17.4197798202338));
#121520=CARTESIAN_POINT('Ctrl Pts',(20.6000283238032,-21.3404499028704,
-17.5469556269153));
#121521=CARTESIAN_POINT('Ctrl Pts',(17.7357373517245,-21.8138571468239,
-17.6741314335968));
#121522=CARTESIAN_POINT('Ctrl Pts',(15.7872904002738,-19.6616880854488,
-17.8013072402782));
#121523=CARTESIAN_POINT('Ctrl Pts',(16.5422666131419,-16.8584242538938,
-17.9284830469596));
#121524=CARTESIAN_POINT('Ctrl Pts',(19.3080221741474,-15.9758862274083,
-18.055658853641));
#121525=CARTESIAN_POINT('Ctrl Pts',(21.5471480181857,-17.8237478688561,
-18.1828346603226));
#121526=CARTESIAN_POINT('Ctrl Pts',(21.2053851592371,-20.7067108133391,
-18.3100104670039));
#121527=CARTESIAN_POINT('Ctrl Pts',(18.5962798080717,-21.9798354963434,
-18.4371862736854));
#121528=CARTESIAN_POINT('Ctrl Pts',(16.1135241852737,-20.4751090398787,
-18.5643620803668));
#121529=CARTESIAN_POINT('Ctrl Pts',(16.0348924771216,-17.5730245745949,
-18.6915378870482));
#121530=CARTESIAN_POINT('Ctrl Pts',(18.4325243962693,-15.9360644723642,
-18.8187136937296));
#121531=CARTESIAN_POINT('Ctrl Pts',(21.1067414690649,-17.0660380283814,
-18.9458895004112));
#121532=CARTESIAN_POINT('Ctrl Pts',(21.6041155150354,-19.9262646340588,
-19.0730653070925));
#121533=CARTESIAN_POINT('Ctrl Pts',(19.4683367113789,-21.8926639140248,
-19.2002411137739));
#121534=CARTESIAN_POINT('Ctrl Pts',(16.6588495608948,-21.1611865588169,
-19.3274169204554));
#121535=CARTESIAN_POINT('Ctrl Pts',(15.7531841249269,-18.4029176770636,
-19.4545927271368));
#121536=CARTESIAN_POINT('Ctrl Pts',(17.582232272941,-16.148397701268,-19.5817685338183));
#121537=CARTESIAN_POINT('Ctrl Pts',(20.4679557680829,-16.4660089109295,
-19.7089443404997));
#121538=CARTESIAN_POINT('Ctrl Pts',(21.762882574719,-19.0643624781199,-19.8361201471812));
#121539=CARTESIAN_POINT('Ctrl Pts',(20.278997406019,-21.5596307706316,-19.9632959538626));
#121540=CARTESIAN_POINT('Ctrl Pts',(17.3776734088588,-21.662559052761,-20.0904717605441));
#121541=CARTESIAN_POINT('Ctrl Pts',(15.7206941087448,-19.2787188466078,
-20.2176475672255));
#121542=CARTESIAN_POINT('Ctrl Pts',(16.828237415124,-16.5951320529376,-20.3448233739069));
#121543=CARTESIAN_POINT('Ctrl Pts',(19.6841967603538,-16.0738297948901,
-20.4719991805884));
#121544=CARTESIAN_POINT('Ctrl Pts',(21.6684150405127,-18.1930614333217,
-20.5991749872697));
#121545=CARTESIAN_POINT('Ctrl Pts',(20.9604790804735,-21.0085887233582,
-20.7263507939513));
#121546=CARTESIAN_POINT('Ctrl Pts',(18.2099071212035,-21.9372914819773,
-20.8535266006326));
#121547=CARTESIAN_POINT('Ctrl Pts',(15.9401186110067,-20.1272362927054,
-20.980702407314));
#121548=CARTESIAN_POINT('Ctrl Pts',(16.2336184655874,-17.2388558767421,
-21.1078782139955));
#121549=CARTESIAN_POINT('Ctrl Pts',(18.8209175351634,-15.9224078905259,
-21.2350540206769));
#121550=CARTESIAN_POINT('Ctrl Pts',(21.3287557911663,-17.3849813380486,
-21.3622298273583));
#121551=CARTESIAN_POINT('Ctrl Pts',(21.4555258683986,-20.286047713047,-21.4894056340398));
#121552=CARTESIAN_POINT('Ctrl Pts',(19.0865078830173,-21.9615659646048,
-21.6165814407212));
#121553=CARTESIAN_POINT('Ctrl Pts',(16.3920659006521,-20.879190353892,-21.7437572474027));
#121554=CARTESIAN_POINT('Ctrl Pts',(15.8501931440795,-18.0222746586101,
-21.8709330540841));
#121555=CARTESIAN_POINT('Ctrl Pts',(17.2469900335074,-16.6964452121458,
-21.9557169252051));
#121556=CARTESIAN_POINT('Ctrl Pts',(18.0714160310384,-16.4758408723594,
-21.9981088607656));
#121557=CARTESIAN_POINT('Ctrl Pts',(20.3539256943887,-17.5890877707427,
0.));
#121558=CARTESIAN_POINT('Ctrl Pts',(20.4076089239479,-17.6408883813468,
-1.14883615034368E-14));
#121559=CARTESIAN_POINT('Ctrl Pts',(20.458135595812,-17.6955615793788,-3.45732861075315E-15));
#121560=CARTESIAN_POINT('Ctrl Pts',(20.505511977026,-17.7527360595703,-3.1641356201817E-15));
#121561=CARTESIAN_POINT('Ctrl Pts',(20.554575660781,-17.811946800093,-2.86050060627935E-15));
#121562=CARTESIAN_POINT('Ctrl Pts',(20.6002611686399,-17.8738405959818,
-1.28830115027514E-14));
#121563=CARTESIAN_POINT('Ctrl Pts',(20.6425471220964,-17.938054648476,-1.24275589818978E-14));
#121564=CARTESIAN_POINT('Ctrl Pts',(20.6826816235517,-17.9990015770096,
-1.19952792680244E-14));
#121565=CARTESIAN_POINT('Ctrl Pts',(20.7197537535955,-18.0620396014581,
-1.56156834274937E-14));
#121566=CARTESIAN_POINT('Ctrl Pts',(20.7537167666138,-18.1268912820608,
-3.64291929955129E-15));
#121567=CARTESIAN_POINT('Ctrl Pts',(20.7688150878339,-18.1557212184648,
1.86923291261623E-15));
#121568=CARTESIAN_POINT('Ctrl Pts',(20.7832985724702,-18.1849099468526,
1.07609079391212E-16));
#121569=CARTESIAN_POINT('Ctrl Pts',(20.7971611207678,-18.2144346312911,
4.69763117294519E-15));
#121570=CARTESIAN_POINT('Ctrl Pts',(20.8057380545325,-18.2327019265545,
7.27018219478905E-15));
#121571=CARTESIAN_POINT('Ctrl Pts',(20.8140776656103,-18.2510987616938,
-4.62727264044915E-15));
#121572=CARTESIAN_POINT('Ctrl Pts',(20.8221770088969,-18.269617013417,-1.43565714871841E-14));
#121573=CARTESIAN_POINT('Ctrl Pts',(20.8264660877165,-18.2794235172817,
-1.95088076791796E-14));
#121574=CARTESIAN_POINT('Ctrl Pts',(20.8306870781385,-18.2892625308288,
-2.33904285261234E-14));
#121575=CARTESIAN_POINT('Ctrl Pts',(20.8348368140281,-18.2991258749815,
-2.39808173319034E-14));
#121576=CARTESIAN_POINT('Ctrl Pts',(20.8659056770803,-18.372972234574,-2.9180491333638E-14));
#121577=CARTESIAN_POINT('Ctrl Pts',(20.8930393303568,-18.4483069573626,
-1.39833664931511E-14));
#121578=CARTESIAN_POINT('Ctrl Pts',(20.9162161420459,-18.5247489058203,
-2.07472927726826E-14));
#121579=CARTESIAN_POINT('Ctrl Pts',(20.9398193164084,-18.6025970871087,
-2.76356488370442E-14));
#121580=CARTESIAN_POINT('Ctrl Pts',(20.9593192432917,-18.681594415105,7.90483084619676E-15));
#121581=CARTESIAN_POINT('Ctrl Pts',(20.9746521798118,-18.7613738906752,
-2.84494650060196E-15));
#121582=CARTESIAN_POINT('Ctrl Pts',(20.9885844406084,-18.8338654488586,
-1.26127232931092E-14));
#121583=CARTESIAN_POINT('Ctrl Pts',(20.9990759862006,-18.9070037360463,
-7.2353415164223E-15));
#121584=CARTESIAN_POINT('Ctrl Pts',(21.0060452061984,-18.9805292501327,
-6.82787160144471E-15));
#121585=CARTESIAN_POINT('Ctrl Pts',(21.0087031403799,-19.0085705484655,
-6.66025088122286E-15));
#121586=CARTESIAN_POINT('Ctrl Pts',(21.0108483899423,-19.0366682762212,
-1.4471649499982E-15));
#121587=CARTESIAN_POINT('Ctrl Pts',(21.0124750673575,-19.0648083237754,
-9.10382880192628E-15));
#121588=CARTESIAN_POINT('Ctrl Pts',(21.0133685834701,-19.0802653441188,
-1.32692796682525E-14));
#121589=CARTESIAN_POINT('Ctrl Pts',(21.014105623128,-19.0957351348357,-1.68888790667805E-14));
#121590=CARTESIAN_POINT('Ctrl Pts',(21.0146851084115,-19.1112153648711,
3.7470027081099E-15));
#121591=CARTESIAN_POINT('Ctrl Pts',(21.0151328224698,-19.1231754901941,
2.01287399453959E-14));
#121592=CARTESIAN_POINT('Ctrl Pts',(21.0154863189935,-19.1351385470168,
-5.6262880174693E-15));
#121593=CARTESIAN_POINT('Ctrl Pts',(21.0157451770828,-19.1470949182306,
-6.38378239159465E-15));
#121594=CARTESIAN_POINT('Ctrl Pts',(21.0175519249061,-19.2305466184455,
-1.17840328135284E-14));
#121595=CARTESIAN_POINT('Ctrl Pts',(21.0147568373932,-19.3137920798114,
1.49690073973068E-14));
#121596=CARTESIAN_POINT('Ctrl Pts',(21.0073036695044,-19.3964506692726,
1.12271303365219E-14));
#121597=CARTESIAN_POINT('Ctrl Pts',(20.9998648261745,-19.4789503936919,
7.57364944833593E-15));
#121598=CARTESIAN_POINT('Ctrl Pts',(20.9877861648147,-19.5608665038776,
8.08948018227706E-15));
#121599=CARTESIAN_POINT('Ctrl Pts',(20.9709624036051,-19.6418361818354,
1.15740750317173E-14));
#121600=CARTESIAN_POINT('Ctrl Pts',(20.9545246825771,-19.7209479191819,
1.49539710127781E-14));
#121601=CARTESIAN_POINT('Ctrl Pts',(20.9335573448041,-19.799157111958,8.98046188800277E-15));
#121602=CARTESIAN_POINT('Ctrl Pts',(20.9083260528412,-19.8762372781696,
1.75970349403087E-14));
#121603=CARTESIAN_POINT('Ctrl Pts',(20.8979286223519,-19.9080008387303,
2.11190768885281E-14));
#121604=CARTESIAN_POINT('Ctrl Pts',(20.886806496403,-19.9395726045308,6.78433755510298E-15));
#121605=CARTESIAN_POINT('Ctrl Pts',(20.8749757808311,-19.9709362516545,
-5.4678483962789E-15));
#121606=CARTESIAN_POINT('Ctrl Pts',(20.8684245113494,-19.9883038997047,
-1.2315661009052E-14));
#121607=CARTESIAN_POINT('Ctrl Pts',(20.8616537141196,-20.0056128698145,
8.27179597674389E-15));
#121608=CARTESIAN_POINT('Ctrl Pts',(20.8546785166995,-20.0228303119358,
5.07927033766009E-15));
#121609=CARTESIAN_POINT('Ctrl Pts',(20.8236218670382,-20.0994899440325,
-8.89802862727266E-15));
#121610=CARTESIAN_POINT('Ctrl Pts',(20.7884837604207,-20.1744320701159,
-3.12356070928148E-15));
#121611=CARTESIAN_POINT('Ctrl Pts',(20.7495952387339,-20.2474309568179,
-1.0325074129014E-14));
#121612=CARTESIAN_POINT('Ctrl Pts',(20.7099066604842,-20.321931655259,-1.76747448410191E-14));
#121613=CARTESIAN_POINT('Ctrl Pts',(20.6663114480309,-20.3944090798955,
1.85848361403515E-14));
#121614=CARTESIAN_POINT('Ctrl Pts',(20.6191066061262,-20.4646182429904,
4.49640324973188E-15));
#121615=CARTESIAN_POINT('Ctrl Pts',(20.5711286079629,-20.5359773443472,
-9.82278054742002E-15));
#121616=CARTESIAN_POINT('Ctrl Pts',(20.5194213554741,-20.6049941328796,
-2.55515037437809E-15));
#121617=CARTESIAN_POINT('Ctrl Pts',(20.4642461984827,-20.6713939738053,
2.77555756156289E-15));
#121618=CARTESIAN_POINT('Ctrl Pts',(20.4403643182492,-20.7001343188262,
5.08288816881304E-15));
#121619=CARTESIAN_POINT('Ctrl Pts',(20.4158321356568,-20.7283840869166,
6.72524383598771E-15));
#121620=CARTESIAN_POINT('Ctrl Pts',(20.3906682941055,-20.7561193805442,
3.1641356201817E-15));
#121621=CARTESIAN_POINT('Ctrl Pts',(20.3815365270621,-20.7661843080224,
1.76576788124933E-15));
#121622=CARTESIAN_POINT('Ctrl Pts',(20.3723208078371,-20.7761822779911,
-4.33283550333587E-16));
#121623=CARTESIAN_POINT('Ctrl Pts',(20.3630243316464,-20.7861096027615,
1.94289029309402E-16));
#121624=CARTESIAN_POINT('Ctrl Pts',(20.3025147033051,-20.8507253474758,
4.82486799989442E-15));
#121625=CARTESIAN_POINT('Ctrl Pts',(20.2387852854453,-20.9121400047012,
1.82120019294766E-14));
#121626=CARTESIAN_POINT('Ctrl Pts',(20.1721441659295,-20.9700792099884,
2.01505478969466E-14));
#121627=CARTESIAN_POINT('Ctrl Pts',(20.1169512585411,-21.0180650964023,
2.17560729665775E-14));
#121628=CARTESIAN_POINT('Ctrl Pts',(20.0597599950038,-21.0636670219304,
1.76866719771448E-14));
#121629=CARTESIAN_POINT('Ctrl Pts',(20.0007222397457,-21.1067151539364,
1.05748743095546E-14));
#121630=CARTESIAN_POINT('Ctrl Pts',(19.9812253420094,-21.1209315655156,
8.41816628900994E-15));
#121631=CARTESIAN_POINT('Ctrl Pts',(19.9615269106471,-21.1348693297411,
-1.5795805565849E-14));
#121632=CARTESIAN_POINT('Ctrl Pts',(19.941631987048,-21.1485219218181,-5.80091530366644E-15));
#121633=CARTESIAN_POINT('Ctrl Pts',(19.9257068710437,-21.1594502931437,
2.07770478644972E-15));
#121634=CARTESIAN_POINT('Ctrl Pts',(19.9096544895287,-21.170196697329,1.40562940309176E-14));
#121635=CARTESIAN_POINT('Ctrl Pts',(19.8934933729568,-21.1807476067171,
1.42941214420489E-14));
#121636=CARTESIAN_POINT('Ctrl Pts',(19.8189655561075,-21.2294036657816,
1.49872222632139E-14));
#121637=CARTESIAN_POINT('Ctrl Pts',(19.7420556060774,-21.2739560343907,
1.33704818268334E-14));
#121638=CARTESIAN_POINT('Ctrl Pts',(19.6630443896218,-21.3141141071315,
1.13797860024079E-14));
#121639=CARTESIAN_POINT('Ctrl Pts',(19.585203146919,-21.3536775315023,9.81319007009315E-15));
#121640=CARTESIAN_POINT('Ctrl Pts',(19.5053217267533,-21.3889765584864,
2.19043743988934E-14));
#121641=CARTESIAN_POINT('Ctrl Pts',(19.4236362626317,-21.4196959407397,
5.55111512312578E-17));
#121642=CARTESIAN_POINT('Ctrl Pts',(19.4149414973774,-21.4229657736325,
-2.15692061228505E-15));
#121643=CARTESIAN_POINT('Ctrl Pts',(19.4062262673531,-21.4261836782215,
3.67808051293056E-14));
#121644=CARTESIAN_POINT('Ctrl Pts',(19.3974909880357,-21.4293497847436,
2.33146835171283E-15));
#121645=CARTESIAN_POINT('Ctrl Pts',(18.0714161019496,-21.428158862637,-0.00189098085166848));
#121646=CARTESIAN_POINT('Ctrl Pts',(17.2469901926503,-21.2075545464601,
-0.0442829164121466));
#121647=CARTESIAN_POINT('Ctrl Pts',(15.8501939821074,-19.8817220316731,
-0.129066787533102));
#121648=CARTESIAN_POINT('Ctrl Pts',(16.3920656827787,-17.0248116182672,
-0.256242594214537));
#121649=CARTESIAN_POINT('Ctrl Pts',(19.0865079334355,-15.9424330181619,
-0.38341840089597));
#121650=CARTESIAN_POINT('Ctrl Pts',(21.4555257912919,-17.6179530146914,
-0.510594207577405));
#121651=CARTESIAN_POINT('Ctrl Pts',(21.3287556480917,-20.5190182015967,
-0.63777001425884));
#121652=CARTESIAN_POINT('Ctrl Pts',(18.8209175719769,-21.9815922294721,
-0.764945820940274));
#121653=CARTESIAN_POINT('Ctrl Pts',(16.2336185304982,-20.6651439233068,
-0.892121627621709));
#121654=CARTESIAN_POINT('Ctrl Pts',(15.9401187363004,-17.7767638289518,
-1.01929743430314));
#121655=CARTESIAN_POINT('Ctrl Pts',(18.2099071283678,-15.9667085869429,
-1.14647324098458));
#121656=CARTESIAN_POINT('Ctrl Pts',(20.9604790041794,-16.8954113789202,
-1.27364904766601));
#121657=CARTESIAN_POINT('Ctrl Pts',(21.6684149250656,-19.7109385242504,
-1.40082485434745));
#121658=CARTESIAN_POINT('Ctrl Pts',(19.6841967272255,-21.8301701041092,
-1.52800066102888));
#121659=CARTESIAN_POINT('Ctrl Pts',(16.8282374854801,-21.3088678538367,
-1.65517646771032));
#121660=CARTESIAN_POINT('Ctrl Pts',(15.720694223426,-18.6252811680681,-1.78235227439175));
#121661=CARTESIAN_POINT('Ctrl Pts',(17.3776734595451,-16.2414410482877,
-1.90952808107318));
#121662=CARTESIAN_POINT('Ctrl Pts',(20.2789973479827,-16.3443693285228,
-2.03670388775462));
#121663=CARTESIAN_POINT('Ctrl Pts',(21.7628824602007,-18.839637525737,-2.16387969443605));
#121664=CARTESIAN_POINT('Ctrl Pts',(20.4679557027106,-21.4379909954235,
-2.29105550111749));
#121665=CARTESIAN_POINT('Ctrl Pts',(17.5822323163742,-21.7556021927696,
-2.41823130779892));
#121666=CARTESIAN_POINT('Ctrl Pts',(15.7531842374939,-19.5010823022681,
-2.54540711448036));
#121667=CARTESIAN_POINT('Ctrl Pts',(16.6588496392251,-16.7428135245559,
-2.67258292116179));
#121668=CARTESIAN_POINT('Ctrl Pts',(19.468336683663,-16.0113361970163,-2.79975872784322));
#121669=CARTESIAN_POINT('Ctrl Pts',(21.6041154066714,-17.977735402714,-2.92693453452466));
#121670=CARTESIAN_POINT('Ctrl Pts',(21.1067413794861,-20.8379619004206,
-3.05411034120609));
#121671=CARTESIAN_POINT('Ctrl Pts',(18.43252440765,-21.9679354137682,-3.18128614788753));
#121672=CARTESIAN_POINT('Ctrl Pts',(16.0348925790254,-20.3309753733442,
-3.30846195456896));
#121673=CARTESIAN_POINT('Ctrl Pts',(16.1135242842076,-17.4288910176245,
-3.43563776125039));
#121674=CARTESIAN_POINT('Ctrl Pts',(18.5962798132715,-15.924164617971,-3.56281356793183));
#121675=CARTESIAN_POINT('Ctrl Pts',(21.2053850659314,-17.1972892529086,
-3.68998937461327));
#121676=CARTESIAN_POINT('Ctrl Pts',(21.5471479119772,-20.0802520885476,
-3.8171651812947));
#121677=CARTESIAN_POINT('Ctrl Pts',(19.3080221524756,-21.9281136602303,
-3.94434098797614));
#121678=CARTESIAN_POINT('Ctrl Pts',(16.5422666958893,-21.0455756670647,
-4.07151679465757));
#121679=CARTESIAN_POINT('Ctrl Pts',(15.7872905115249,-18.242311941345,-4.198692601339));
#121680=CARTESIAN_POINT('Ctrl Pts',(17.7357373894132,-16.0901429612237,
-4.32586840802044));
#121681=CARTESIAN_POINT('Ctrl Pts',(20.6000282533525,-16.5635501873038,
-4.45304421470187));
#121682=CARTESIAN_POINT('Ctrl Pts',(21.7523540136147,-19.2282118726162,
-4.5802200213833));
#121683=CARTESIAN_POINT('Ctrl Pts',(20.1355273065643,-21.6394663084466,
-4.70739582806474));
#121684=CARTESIAN_POINT('Ctrl Pts',(17.2328862843358,-21.5851372092476,
-4.83457163474617));
#121685=CARTESIAN_POINT('Ctrl Pts',(15.7074239266047,-19.115068151491,-4.96174744142761));
#121686=CARTESIAN_POINT('Ctrl Pts',(16.9586572657169,-16.4953941858922,
-5.08892324810904));
#121687=CARTESIAN_POINT('Ctrl Pts',(19.8386573733367,-16.1295035805846,
-5.21609905479048));
#121688=CARTESIAN_POINT('Ctrl Pts',(21.705202903689,-18.3530782562058,-5.34327486147191));
#121689=CARTESIAN_POINT('Ctrl Pts',(20.8458541835569,-21.1261264584823,
-5.47045066815334));
#121690=CARTESIAN_POINT('Ctrl Pts',(18.0490103264645,-21.9045485766079,
-5.59762647483478));
#121691=CARTESIAN_POINT('Ctrl Pts',(15.8806019795871,-19.9741906315278,
-5.72480228151621));
#121692=CARTESIAN_POINT('Ctrl Pts',(16.3300092145838,-17.1060362263267,
-5.85197808819766));
#121693=CARTESIAN_POINT('Ctrl Pts',(18.9849287867042,-15.9314390100375,
-5.97915389487907));
#121694=CARTESIAN_POINT('Ctrl Pts',(21.4096367714204,-17.5280190248805,
-6.10632970156052));
#121695=CARTESIAN_POINT('Ctrl Pts',(21.3796140871054,-20.4310132021685,
-6.23350550824194));
#121696=CARTESIAN_POINT('Ctrl Pts',(18.9224046832003,-21.9771045643792,
-6.36068131492339));
#121697=CARTESIAN_POINT('Ctrl Pts',(16.2923456761723,-20.7478502479364,
-6.48785712160482));
#121698=CARTESIAN_POINT('Ctrl Pts',(15.9023529650977,-17.8710147920491,
-6.61503292828625));
#121699=CARTESIAN_POINT('Ctrl Pts',(18.1102206567097,-15.9859161709479,
-6.74220873496769));
#121700=CARTESIAN_POINT('Ctrl Pts',(20.8903671796782,-16.8220153670774,
-6.86938454164913));
#121701=CARTESIAN_POINT('Ctrl Pts',(21.6921806545333,-19.6122432621575,
-6.99656034833056));
#121702=CARTESIAN_POINT('Ctrl Pts',(19.7800469842523,-21.7967389435265,
-7.12373615501199));
#121703=CARTESIAN_POINT('Ctrl Pts',(16.9082301309179,-21.3713632086215,
-7.25091196169343));
#121704=CARTESIAN_POINT('Ctrl Pts',(15.711443812408,-18.7263718924222,-7.37808776837486));
#121705=CARTESIAN_POINT('Ctrl Pts',(17.2876651950193,-16.2883803608658,
-7.5052635750563));
#121706=CARTESIAN_POINT('Ctrl Pts',(20.1908089915383,-16.2940945253353,
-7.63243938173773));
#121707=CARTESIAN_POINT('Ctrl Pts',(21.7574209580843,-18.7382719945909,
-7.75961518841917));
#121708=CARTESIAN_POINT('Ctrl Pts',(20.5502318502561,-21.3785316433533,
-7.8867909951006));
#121709=CARTESIAN_POINT('Ctrl Pts',(17.6767627478799,-21.7925991168782,
-8.01396680178203));
#121710=CARTESIAN_POINT('Ctrl Pts',(15.7732432047795,-19.6005932081323,
-8.14114260846348));
#121711=CARTESIAN_POINT('Ctrl Pts',(16.5860342560023,-16.8135432871596,
-8.26831841514489));
#121712=CARTESIAN_POINT('Ctrl Pts',(19.3694505595535,-15.9883946726254,
-8.39549422182634));
#121713=CARTESIAN_POINT('Ctrl Pts',(21.5698804152241,-17.8821700038661,
-8.52267002850777));
#121714=CARTESIAN_POINT('Ctrl Pts',(21.1685660045158,-20.7574479554213,
-8.6498458351892));
#121715=CARTESIAN_POINT('Ctrl Pts',(18.5336883908723,-21.9763394666155,
-8.77702164187065));
#121716=CARTESIAN_POINT('Ctrl Pts',(16.0825842458626,-20.4205872288672,
-8.90419744855206));
#121717=CARTESIAN_POINT('Ctrl Pts',(16.0639894898528,-17.5174973594366,
-9.03137325523352));
#121718=CARTESIAN_POINT('Ctrl Pts',(18.4949636573611,-15.9304746274477,
-9.15854906191495));
#121719=CARTESIAN_POINT('Ctrl Pts',(21.1452388329719,-17.1155138877607,
-9.28572486859637));
#121720=CARTESIAN_POINT('Ctrl Pts',(21.5833520376912,-19.98541517087,-9.4129006752778));
#121721=CARTESIAN_POINT('Ctrl Pts',(19.4073615985613,-21.9072221756853,
-9.54007648195925));
#121722=CARTESIAN_POINT('Ctrl Pts',(16.6136036862856,-21.1177962560837,
-9.66725228864067));
#121723=CARTESIAN_POINT('Ctrl Pts',(15.7651777852051,-18.3413866960012,
-9.79442809532212));
#121724=CARTESIAN_POINT('Ctrl Pts',(17.6404620003109,-16.1251769434017,
-9.92160390200354));
#121725=CARTESIAN_POINT('Ctrl Pts',(20.5189994575086,-16.5024018928049,
-10.048779708685));
#121726=CARTESIAN_POINT('Ctrl Pts',(21.7599107020031,-19.1269810663543,
-10.1759555153665));
#121727=CARTESIAN_POINT('Ctrl Pts',(20.2247366866089,-21.5910259720733,
-10.3031313220479));
#121728=CARTESIAN_POINT('Ctrl Pts',(17.3219042868047,-21.6339283448398,
-10.4303071287293));
#121729=CARTESIAN_POINT('Ctrl Pts',(15.7145820593127,-19.2163279204619,
-10.5574829354107));
#121730=CARTESIAN_POINT('Ctrl Pts',(16.8773883861884,-16.5562230351012,
-10.6846587420922));
#121731=CARTESIAN_POINT('Ctrl Pts',(19.7435206344235,-16.0940948163466,
-10.8118345487736));
#121732=CARTESIAN_POINT('Ctrl Pts',(21.683480358492,-18.2539172219934,-10.9390103554551));
#121733=CARTESIAN_POINT('Ctrl Pts',(20.9174749190411,-21.0541872485576,
-11.0661861621365));
#121734=CARTESIAN_POINT('Ctrl Pts',(18.1482667631075,-21.9258309510259,
-11.1933619688179));
#121735=CARTESIAN_POINT('Ctrl Pts',(15.9164324973179,-20.069169332693,-11.3205377754993));
#121736=CARTESIAN_POINT('Ctrl Pts',(16.2695415372774,-17.1875741909633,
-11.4477135821808));
#121737=CARTESIAN_POINT('Ctrl Pts',(18.8836382552418,-15.9247302164082,
-11.5748893888622));
#121738=CARTESIAN_POINT('Ctrl Pts',(21.3604511616193,-17.4392183747454,
-11.7020651955437));
#121739=CARTESIAN_POINT('Ctrl Pts',(21.427658143155,-20.3415897804367,-11.8292410022251));
#121740=CARTESIAN_POINT('Ctrl Pts',(19.0236009656254,-21.9690988102461,
-11.9564168089065));
#121741=CARTESIAN_POINT('Ctrl Pts',(16.3538528767977,-20.8286069439261,
-12.083592615588));
#121742=CARTESIAN_POINT('Ctrl Pts',(15.8677420449167,-17.9664446819167,
-12.2107684222694));
#121743=CARTESIAN_POINT('Ctrl Pts',(18.0112449867927,-16.008468253787,-12.3379442289508));
#121744=CARTESIAN_POINT('Ctrl Pts',(20.817830794051,-16.7509995066233,-12.4651200356323));
#121745=CARTESIAN_POINT('Ctrl Pts',(21.712631184893,-19.5128121026353,-12.5922958423137));
#121746=CARTESIAN_POINT('Ctrl Pts',(19.874722338297,-21.7601144024042,-12.7194716489951));
#121747=CARTESIAN_POINT('Ctrl Pts',(16.9902715475267,-21.4311460292034,
-12.8466474556766));
#121748=CARTESIAN_POINT('Ctrl Pts',(15.7055833839069,-18.8277150473647,
-12.973823262358));
#121749=CARTESIAN_POINT('Ctrl Pts',(17.1992795008189,-16.3383077955748,
-13.1009990690394));
#121750=CARTESIAN_POINT('Ctrl Pts',(20.1009864202325,-16.2468009173113,
-13.2281748757209));
#121751=CARTESIAN_POINT('Ctrl Pts',(21.7485681438287,-18.6371462938237,
-13.3553506824023));
#121752=CARTESIAN_POINT('Ctrl Pts',(20.6304707006625,-21.3163504037278,
-13.4825264890837));
#121753=CARTESIAN_POINT('Ctrl Pts',(17.7724790978853,-21.8264097663479,
-13.6097022957652));
#121754=CARTESIAN_POINT('Ctrl Pts',(15.7966232440805,-19.6993765743343,
-13.7368781024466));
#121755=CARTESIAN_POINT('Ctrl Pts',(16.5156282496692,-16.8866717627907,
-13.864053909128));
#121756=CARTESIAN_POINT('Ctrl Pts',(19.2698516485073,-15.9687774201593,
-13.9912297158095));
#121757=CARTESIAN_POINT('Ctrl Pts',(21.532464418544,-17.7878046348562,-14.1184055224909));
#121758=CARTESIAN_POINT('Ctrl Pts',(21.2276597768573,-20.674908838959,-14.2455813291723));
#121759=CARTESIAN_POINT('Ctrl Pts',(18.6350770638849,-21.9813511190996,
-14.3727571358538));
#121760=CARTESIAN_POINT('Ctrl Pts',(16.1332500049482,-20.5085517702016,
-14.4999329425352));
#121761=CARTESIAN_POINT('Ctrl Pts',(16.0174496457219,-17.6077127826422,
-14.6271087492167));
#121762=CARTESIAN_POINT('Ctrl Pts',(18.3939156284153,-15.940173881134,-14.7542845558981));
#121763=CARTESIAN_POINT('Ctrl Pts',(21.082387914021,-17.0357985086741,-14.8814603625795));
#121764=CARTESIAN_POINT('Ctrl Pts',(21.6163600459046,-19.889419071628,-15.008636169261));
#121765=CARTESIAN_POINT('Ctrl Pts',(19.5059457351114,-21.8830158191527,
-15.1358119759424));
#121766=CARTESIAN_POINT('Ctrl Pts',(16.6873191247092,-21.1875874719632,
-15.2629877826238));
#121767=CARTESIAN_POINT('Ctrl Pts',(15.7463951860447,-18.4411463754548,
-15.3901635893052));
#121768=CARTESIAN_POINT('Ctrl Pts',(17.5464132325167,-16.1633817723147,
-15.5173393959867));
#121769=CARTESIAN_POINT('Ctrl Pts',(20.4359684282068,-16.4440013119089,
-15.6445152026681));
#121770=CARTESIAN_POINT('Ctrl Pts',(21.7640732270913,-19.0255539838723,
-15.7716910093496));
#121771=CARTESIAN_POINT('Ctrl Pts',(20.3122739076741,-21.539625440908,-15.898866816031));
#121772=CARTESIAN_POINT('Ctrl Pts',(17.4125062366922,-21.6797111620585,
-16.0260426227124));
#121773=CARTESIAN_POINT('Ctrl Pts',(15.725127072392,-19.3172911928685,-16.1532184293939));
#121774=CARTESIAN_POINT('Ctrl Pts',(16.7982020674565,-16.6197392267502,
-16.2803942360753));
#121775=CARTESIAN_POINT('Ctrl Pts',(19.6472515164596,-16.0618917636594,
-16.4075700427567));
#121776=CARTESIAN_POINT('Ctrl Pts',(21.6584493818927,-18.1555392270637,
-16.5347458494382));
#121777=CARTESIAN_POINT('Ctrl Pts',(20.9866464512386,-20.9798900157063,
-16.6619216561196));
#121778=CARTESIAN_POINT('Ctrl Pts',(18.24818021658,-21.9437775799877,-16.789097462801));
#121779=CARTESIAN_POINT('Ctrl Pts',(15.9554234798327,-20.162894905289,-16.9162732694825));
#121780=CARTESIAN_POINT('Ctrl Pts',(16.2118382424305,-17.2710913116015,
-17.0434490761639));
#121781=CARTESIAN_POINT('Ctrl Pts',(18.7821798745847,-15.9214171105603,
-17.1706248828453));
#121782=CARTESIAN_POINT('Ctrl Pts',(21.3083194621878,-17.3521146113923,
-17.2978006895268));
#121783=CARTESIAN_POINT('Ctrl Pts',(21.4726807235191,-20.2506076561855,
-17.4249764962082));
#121784=CARTESIAN_POINT('Ctrl Pts',(19.1244724027178,-21.9577087771101,
-17.5521523028896));
#121785=CARTESIAN_POINT('Ctrl Pts',(16.4180298878732,-20.9072586503617,
-17.6793281095711));
#121786=CARTESIAN_POINT('Ctrl Pts',(15.8363462055885,-18.0629800689462,
-17.8065039162525));
#121787=CARTESIAN_POINT('Ctrl Pts',(17.9130800309984,-16.0343220954698,
-17.9336797229339));
#121788=CARTESIAN_POINT('Ctrl Pts',(20.7429569759279,-16.6824525078913,
-18.0608555296154));
#121789=CARTESIAN_POINT('Ctrl Pts',(21.7297405853753,-19.412751880308,-18.1880313362968));
#121790=CARTESIAN_POINT('Ctrl Pts',(19.9681181443722,-21.7203400000494,
-18.3152071429782));
#121791=CARTESIAN_POINT('Ctrl Pts',(17.0742689039165,-21.4881479922645,
-18.4423829496597));
#121792=CARTESIAN_POINT('Ctrl Pts',(15.7031199295909,-18.9291976127498,
-18.5695587563411));
#121793=CARTESIAN_POINT('Ctrl Pts',(17.1126153022265,-16.3911670081152,
-18.6967345630226));
#121794=CARTESIAN_POINT('Ctrl Pts',(20.0096305005975,-16.2025417305957,
-18.823910369704));
#121795=CARTESIAN_POINT('Ctrl Pts',(21.7363338892051,-18.5363737640858,
-18.9510861763854));
#121796=CARTESIAN_POINT('Ctrl Pts',(20.7085822803688,-21.2515170733997,
-19.0782619830668));
#121797=CARTESIAN_POINT('Ctrl Pts',(17.8692739856059,-21.8569961899794,
-19.2054377897483));
#121798=CARTESIAN_POINT('Ctrl Pts',(15.8232981382665,-19.7973216105359,
-19.3326135964297));
#121799=CARTESIAN_POINT('Ctrl Pts',(16.4477105902148,-16.9621169125157,
-19.4597894031112));
#121800=CARTESIAN_POINT('Ctrl Pts',(19.1696516731346,-15.9525064556156,
-19.5869652097926));
#121801=CARTESIAN_POINT('Ctrl Pts',(21.4919093843545,-17.6947451283222,
-19.714141016474));
#121802=CARTESIAN_POINT('Ctrl Pts',(21.2839564128859,-20.5904371653283,
-19.8413168231554));
#121803=CARTESIAN_POINT('Ctrl Pts',(18.7365766963153,-21.9829646927876,
-19.9684926298369));
#121804=CARTESIAN_POINT('Ctrl Pts',(16.1868330293274,-20.5947704364421,
-20.0956684365183));
#121805=CARTESIAN_POINT('Ctrl Pts',(15.9739569464928,-17.6994358831224,
-20.2228442431997));
#121806=CARTESIAN_POINT('Ctrl Pts',(18.2932490893143,-15.9532519029135,
-20.3500200498812));
#121807=CARTESIAN_POINT('Ctrl Pts',(21.0169027756026,-16.9582317548374,
-20.4771958565626));
#121808=CARTESIAN_POINT('Ctrl Pts',(21.6461349757523,-19.7923729679124,
-20.6043716632441));
#121809=CARTESIAN_POINT('Ctrl Pts',(19.6036638566053,-21.855518855653,-20.7315474699255));
#121810=CARTESIAN_POINT('Ctrl Pts',(16.7633305629729,-21.2548765937423,
-20.8587232766069));
#121811=CARTESIAN_POINT('Ctrl Pts',(15.7309633230734,-18.5414683575651,
-20.9858990832884));
#121812=CARTESIAN_POINT('Ctrl Pts',(17.4536974658068,-16.2047352548569,
-21.1130748899698));
#121813=CARTESIAN_POINT('Ctrl Pts',(20.3510265953171,-16.3883741373928,
-21.2402506966512));
#121814=CARTESIAN_POINT('Ctrl Pts',(21.7648402074573,-18.9241211217718,
-21.3674265033327));
#121815=CARTESIAN_POINT('Ctrl Pts',(20.3980344426769,-21.4851745132897,
-21.4946023100141));
#121816=CARTESIAN_POINT('Ctrl Pts',(17.5046027271422,-21.7227192681557,
-21.6217781166956));
#121817=CARTESIAN_POINT('Ctrl Pts',(15.7390234877918,-19.4172952643212,
-21.748953923377));
#121818=CARTESIAN_POINT('Ctrl Pts',(16.7212336413073,-16.6869333681719,
-21.8761297300584));
#121819=CARTESIAN_POINT('Ctrl Pts',(19.5498595326579,-16.0308555962028,
-22.0033055367398));
#121820=CARTESIAN_POINT('Ctrl Pts',(21.6307164666946,-18.0626227175078,
-22.1305000010223));
#121821=CARTESIAN_POINT('Ctrl Pts',(21.244679026905,-19.9500078602896,-22.2153025297443));
#121822=CARTESIAN_POINT('Ctrl Pts',(20.6946893042483,-20.6030837310341,
-22.2577131229058));
#121823=CARTESIAN_POINT('Ctrl Pts',(18.1101968702393,-21.2832302832024,
0.0847274181292425));
#121824=CARTESIAN_POINT('Ctrl Pts',(17.3340242768668,-21.0755378486675,
0.0423354825687643));
#121825=CARTESIAN_POINT('Ctrl Pts',(16.0189819851084,-19.8273057761765,
-0.0424483885521918));
#121826=CARTESIAN_POINT('Ctrl Pts',(16.5291381537116,-17.1376091768898,
-0.169624195233626));
#121827=CARTESIAN_POINT('Ctrl Pts',(19.0658757862808,-16.118581759655,-0.29680000191506));
#121828=CARTESIAN_POINT('Ctrl Pts',(21.2962359844956,-17.6960342466338,
-0.423975808596494));
#121829=CARTESIAN_POINT('Ctrl Pts',(21.1768856466422,-20.4273012583374,
-0.551151615277929));
#121830=CARTESIAN_POINT('Ctrl Pts',(18.8158303215486,-21.8042714183123,
-0.678327421959364));
#121831=CARTESIAN_POINT('Ctrl Pts',(16.379964849342,-20.5648743004978,-0.805503228640797));
#121832=CARTESIAN_POINT('Ctrl Pts',(16.103643479711,-17.8455499279943,-0.932679035322232));
#121833=CARTESIAN_POINT('Ctrl Pts',(18.2405820727437,-16.1414364891873,
-1.05985484200366));
#121834=CARTESIAN_POINT('Ctrl Pts',(20.8301640861484,-17.0157826813563,
-1.1870306486851));
#121835=CARTESIAN_POINT('Ctrl Pts',(21.4966648031415,-19.6665181585552,
-1.31420645536653));
#121836=CARTESIAN_POINT('Ctrl Pts',(19.6285820960571,-21.6617119688685,
-1.44138226204797));
#121837=CARTESIAN_POINT('Ctrl Pts',(16.9397809967372,-21.1709213290295,
-1.5685580687294));
#121838=CARTESIAN_POINT('Ctrl Pts',(15.897061795067,-18.6444038895142,-1.69573387541083));
#121839=CARTESIAN_POINT('Ctrl Pts',(17.4570587048633,-16.400088970387,-1.82290968209227));
#121840=CARTESIAN_POINT('Ctrl Pts',(20.188569276403,-16.4969928998977,-1.9500854887737));
#121841=CARTESIAN_POINT('Ctrl Pts',(21.58560319155,-18.8462140560325,-2.07726129545514));
#121842=CARTESIAN_POINT('Ctrl Pts',(20.3664679748478,-21.2924869452229,
-2.20443710213657));
#121843=CARTESIAN_POINT('Ctrl Pts',(17.6496448143142,-21.5915084873017,
-2.33161290881801));
#121844=CARTESIAN_POINT('Ctrl Pts',(15.9276501817169,-19.4689447365969,
-2.45878871549944));
#121845=CARTESIAN_POINT('Ctrl Pts',(16.7803073527985,-16.8721163178553,
-2.58596452218088));
#121846=CARTESIAN_POINT('Ctrl Pts',(19.4253562537739,-16.1834520632443,
-2.71314032886231));
#121847=CARTESIAN_POINT('Ctrl Pts',(21.4361287096228,-18.034758716609,-2.84031613554374));
#121848=CARTESIAN_POINT('Ctrl Pts',(20.9678657836256,-20.72757731112,-2.96749194222518));
#121849=CARTESIAN_POINT('Ctrl Pts',(18.4501696524655,-21.7914139305229,
-3.09466774890661));
#121850=CARTESIAN_POINT('Ctrl Pts',(16.1928702476498,-20.2502645009728,
-3.22184355558806));
#121851=CARTESIAN_POINT('Ctrl Pts',(16.2668996708449,-17.5180379719942,
-3.34901936226947));
#121852=CARTESIAN_POINT('Ctrl Pts',(18.6043405202493,-16.1013826015585,
-3.47619516895092));
#121853=CARTESIAN_POINT('Ctrl Pts',(21.0607358948925,-17.2999917651471,
-3.60337097563235));
#121854=CARTESIAN_POINT('Ctrl Pts',(21.3824954994144,-20.0142159489022,
-3.73054678231378));
#121855=CARTESIAN_POINT('Ctrl Pts',(19.2744248674316,-21.7539229281569,
-3.85772258899522));
#121856=CARTESIAN_POINT('Ctrl Pts',(16.6705479621107,-20.9230395277464,
-3.98489839567665));
#121857=CARTESIAN_POINT('Ctrl Pts',(15.9597602292861,-18.2838496971548,
-4.11207420235809));
#121858=CARTESIAN_POINT('Ctrl Pts',(17.7941652973467,-16.2576462993305,
-4.23925000903952));
#121859=CARTESIAN_POINT('Ctrl Pts',(20.4908103723742,-16.7033451914242,
-4.36642581572096));
#121860=CARTESIAN_POINT('Ctrl Pts',(21.5756909706959,-19.2120453031261,
-4.49360162240239));
#121861=CARTESIAN_POINT('Ctrl Pts',(20.053496478638,-21.4821699894429,-4.62077742908383));
#121862=CARTESIAN_POINT('Ctrl Pts',(17.320745864617,-21.4310207505056,-4.74795323576526));
#121863=CARTESIAN_POINT('Ctrl Pts',(15.8845682033658,-19.1055238383603,
-4.8751290424467));
#121864=CARTESIAN_POINT('Ctrl Pts',(17.0625673598435,-16.6391783332833,
-5.00230484912813));
#121865=CARTESIAN_POINT('Ctrl Pts',(19.7740022228553,-16.294703157517,-5.12948065580956));
#121866=CARTESIAN_POINT('Ctrl Pts',(21.5312995962151,-18.388132904286,-5.256656462491));
#121867=CARTESIAN_POINT('Ctrl Pts',(20.7222482100412,-20.9988757138337,
-5.38383226917243));
#121868=CARTESIAN_POINT('Ctrl Pts',(18.0891024957557,-21.7317370993736,
-5.51100807585386));
#121869=CARTESIAN_POINT('Ctrl Pts',(16.0476102147611,-19.9143622261804,
-5.6381838825353));
#121870=CARTESIAN_POINT('Ctrl Pts',(16.4707138255686,-17.2140797414027,
-5.76535968921673));
#121871=CARTESIAN_POINT('Ctrl Pts',(18.9702420260344,-16.1082312263917,
-5.89253549589816));
#121872=CARTESIAN_POINT('Ctrl Pts',(21.2530328304472,-17.6113640569702,
-6.01971130257962));
#121873=CARTESIAN_POINT('Ctrl Pts',(21.2247673617351,-20.3444471560277,
-6.14688710926103));
#121874=CARTESIAN_POINT('Ctrl Pts',(18.9113774330884,-21.8000464144471,
-6.27406291594248));
#121875=CARTESIAN_POINT('Ctrl Pts',(16.4352547188683,-20.6427398573077,
-6.4012387226239));
#121876=CARTESIAN_POINT('Ctrl Pts',(16.0680881238634,-17.934284420239,-6.52841452930535));
#121877=CARTESIAN_POINT('Ctrl Pts',(18.1467302100618,-16.1595198610482,
-6.65559033598677));
#121878=CARTESIAN_POINT('Ctrl Pts',(20.7641558784545,-16.9466825084813,
-6.78276614266821));
#121879=CARTESIAN_POINT('Ctrl Pts',(21.5190395340498,-19.5735994903424,
-6.90994194934964));
#121880=CARTESIAN_POINT('Ctrl Pts',(19.7188222762027,-21.6302375206298,
-7.03711775603107));
#121881=CARTESIAN_POINT('Ctrl Pts',(17.0150917049037,-21.2297588559072,
-7.16429356271251));
#121882=CARTESIAN_POINT('Ctrl Pts',(15.8883528068746,-18.7395778145483,
-7.29146936939396));
#121883=CARTESIAN_POINT('Ctrl Pts',(17.3723185877541,-16.4442809439337,
-7.41864517607538));
#121884=CARTESIAN_POINT('Ctrl Pts',(20.1055425488892,-16.4496606606615,
-7.54582098275682));
#121885=CARTESIAN_POINT('Ctrl Pts',(21.5804613489495,-18.7507814085371,
-7.67299678943824));
#121886=CARTESIAN_POINT('Ctrl Pts',(20.4439285326649,-21.2365077250456,
-7.80017259611969));
#121887=CARTESIAN_POINT('Ctrl Pts',(17.7386424177941,-21.6263399963654,
-7.92734840280111));
#121888=CARTESIAN_POINT('Ctrl Pts',(15.9465351057383,-19.5626313092801,
-8.05452420948257));
#121889=CARTESIAN_POINT('Ctrl Pts',(16.7117538245844,-16.9387062959837,
-8.18170001616398));
#121890=CARTESIAN_POINT('Ctrl Pts',(19.3322578946213,-16.1618532970222,
-8.30887582284543));
#121891=CARTESIAN_POINT('Ctrl Pts',(21.4038974784157,-17.9447867220078,
-8.43605162952684));
#121892=CARTESIAN_POINT('Ctrl Pts',(21.0260718382901,-20.6517758148449,
-8.5632274362083));
#121893=CARTESIAN_POINT('Ctrl Pts',(18.5454125485558,-21.799326097547,-8.69040324288972));
#121894=CARTESIAN_POINT('Ctrl Pts',(16.2377705404641,-20.3346314107382,
-8.81757904957117));
#121895=CARTESIAN_POINT('Ctrl Pts',(16.2202641280231,-17.6014582203607,
-8.94475485625259));
#121896=CARTESIAN_POINT('Ctrl Pts',(18.5089543580768,-16.1073232887258,
-9.07193066293403));
#121897=CARTESIAN_POINT('Ctrl Pts',(21.0041099966872,-17.223002679136,-9.19910646961547));
#121898=CARTESIAN_POINT('Ctrl Pts',(21.4165806122538,-19.9249297977624,
-9.32628227629688));
#121899=CARTESIAN_POINT('Ctrl Pts',(19.3679500158079,-21.7342542137755,
-9.45345808297835));
#121900=CARTESIAN_POINT('Ctrl Pts',(16.7377096272338,-20.9910330748214,
-9.58063388965975));
#121901=CARTESIAN_POINT('Ctrl Pts',(15.9389417519183,-18.3771256463843,
-9.70780969634122));
#121902=CARTESIAN_POINT('Ctrl Pts',(17.7044663383378,-16.2906297566631,
-9.83498550302262));
#121903=CARTESIAN_POINT('Ctrl Pts',(20.4145241592668,-16.6457758819371,
-9.96216130970408));
#121904=CARTESIAN_POINT('Ctrl Pts',(21.5828053691612,-19.1167394951217,
-10.0893371163855));
#121905=CARTESIAN_POINT('Ctrl Pts',(20.1374844696525,-21.4365648464185,
-10.2165129230669));
#121906=CARTESIAN_POINT('Ctrl Pts',(17.4045536793081,-21.4769561606121,
-10.3436887297484));
#121907=CARTESIAN_POINT('Ctrl Pts',(15.8913073734538,-19.2008569138979,
-10.4708645364298));
#121908=CARTESIAN_POINT('Ctrl Pts',(16.9860551150528,-16.6964468944843,
-10.5980403431112));
#121909=CARTESIAN_POINT('Ctrl Pts',(19.6844337988958,-16.2613668539671,
-10.7252161497927));
#121910=CARTESIAN_POINT('Ctrl Pts',(21.5108484628264,-18.294775725408,-10.8523919564741));
#121911=CARTESIAN_POINT('Ctrl Pts',(20.7896770127668,-20.9311470768482,
-10.9795677631555));
#121912=CARTESIAN_POINT('Ctrl Pts',(18.1825494931985,-21.7517738250013,
-11.106743569837));
#121913=CARTESIAN_POINT('Ctrl Pts',(16.081343586742,-20.0037818622775,-11.2339193765184));
#121914=CARTESIAN_POINT('Ctrl Pts',(16.4137852970245,-17.2908453218587,
-11.3610951831999));
#121915=CARTESIAN_POINT('Ctrl Pts',(18.8748799885214,-16.1019150957474,
-11.4882709898813));
#121916=CARTESIAN_POINT('Ctrl Pts',(21.206726034548,-17.5277608730685,-11.6154467965627));
#121917=CARTESIAN_POINT('Ctrl Pts',(21.2699994185634,-20.2602576510996,
-11.7426226032442));
#121918=CARTESIAN_POINT('Ctrl Pts',(19.0066507379223,-21.7925092338742,
-11.8697984099256));
#121919=CARTESIAN_POINT('Ctrl Pts',(16.4931619278508,-20.7187698964554,
-11.996974216607));
#121920=CARTESIAN_POINT('Ctrl Pts',(16.0355029668799,-18.0241288371456,
-12.1241500232885));
#121921=CARTESIAN_POINT('Ctrl Pts',(18.0535475461816,-16.1807519795754,
-12.2513258299699));
#121922=CARTESIAN_POINT('Ctrl Pts',(20.6958650182194,-16.8798231776942,
-12.3785016366513));
#121923=CARTESIAN_POINT('Ctrl Pts',(21.5382931031166,-19.4799879964801,
-12.5056774433328));
#121924=CARTESIAN_POINT('Ctrl Pts',(19.8079563199639,-21.5957565991263,
-12.6328532500142));
#121925=CARTESIAN_POINT('Ctrl Pts',(17.092331270491,-21.2860426121147,-12.7600290566956));
#121926=CARTESIAN_POINT('Ctrl Pts',(15.8828353868898,-18.8349893955103,
-12.8872048633771));
#121927=CARTESIAN_POINT('Ctrl Pts',(17.2891060725835,-16.491286146028,-13.0143806700585));
#121928=CARTESIAN_POINT('Ctrl Pts',(20.0209772564507,-16.4051351284387,
-13.1415564767399));
#121929=CARTESIAN_POINT('Ctrl Pts',(21.5721266863414,-18.6555745542452,
-13.2687322834214));
#121930=CARTESIAN_POINT('Ctrl Pts',(20.5194710355226,-21.1779659282937,
-13.3959080901028));
#121931=CARTESIAN_POINT('Ctrl Pts',(17.8287565284422,-21.6581717221597,
-13.5230838967842));
#121932=CARTESIAN_POINT('Ctrl Pts',(15.9685467207697,-19.6556329249039,
-13.6502597034657));
#121933=CARTESIAN_POINT('Ctrl Pts',(16.6454686534027,-17.0075545914336,
-13.7774355101471));
#121934=CARTESIAN_POINT('Ctrl Pts',(19.2384884676639,-16.14338423443,-13.9046113168286));
#121935=CARTESIAN_POINT('Ctrl Pts',(21.3686714249291,-17.8559445199825,
-14.03178712351));
#121936=CARTESIAN_POINT('Ctrl Pts',(21.0817068759728,-20.5740676795759,
-14.1589629301914));
#121937=CARTESIAN_POINT('Ctrl Pts',(18.6408669834337,-21.8040444200327,
-14.2861387368729));
#121938=CARTESIAN_POINT('Ctrl Pts',(16.2854708531072,-20.4174474229502,
-14.4133145435543));
#121939=CARTESIAN_POINT('Ctrl Pts',(16.1764482421967,-17.6863933712359,
-14.5404903502357));
#121940=CARTESIAN_POINT('Ctrl Pts',(18.413820629506,-16.1164548490061,-14.6676661569172));
#121941=CARTESIAN_POINT('Ctrl Pts',(20.9449377166707,-17.1479530090328,
-14.7948419635986));
#121942=CARTESIAN_POINT('Ctrl Pts',(21.4476566750608,-19.8345523114875,
-14.92201777028));
#121943=CARTESIAN_POINT('Ctrl Pts',(19.4607640626112,-21.7114646455266,
-15.0491935769614));
#121944=CARTESIAN_POINT('Ctrl Pts',(16.8071105307807,-21.0567394389867,
-15.1763693836429));
#121945=CARTESIAN_POINT('Ctrl Pts',(15.9212584907105,-18.471046432039,-15.3035451903243));
#121946=CARTESIAN_POINT('Ctrl Pts',(17.6159222069866,-16.3265984723504,
-15.4307209970058));
#121947=CARTESIAN_POINT('Ctrl Pts',(20.3363529026182,-16.5907934634841,
-15.5578968036872));
#121948=CARTESIAN_POINT('Ctrl Pts',(21.5867242633349,-19.0212488988654,
-15.6850726103686));
#121949=CARTESIAN_POINT('Ctrl Pts',(20.2198981724784,-21.388172767609,-15.8122484170501));
#121950=CARTESIAN_POINT('Ctrl Pts',(17.4898527336144,-21.5200593280063,
-15.9394242237315));
#121951=CARTESIAN_POINT('Ctrl Pts',(15.9012351911711,-19.2959108466956,
-16.0666000304129));
#121952=CARTESIAN_POINT('Ctrl Pts',(16.9115035396152,-16.7562455090563,
-16.1937758370943));
#121953=CARTESIAN_POINT('Ctrl Pts',(19.5937992735749,-16.2310486329641,
-16.3209516437758));
#121954=CARTESIAN_POINT('Ctrl Pts',(21.4872825391909,-18.2021557548393,
-16.4481274504572));
#121955=CARTESIAN_POINT('Ctrl Pts',(20.8547999630863,-20.8611984310668,
-16.5753032571387));
#121956=CARTESIAN_POINT('Ctrl Pts',(18.2766150525408,-21.7686700450093,
-16.7024790638201));
#121957=CARTESIAN_POINT('Ctrl Pts',(16.1180524427778,-20.092021714915,-16.8296548705015));
#121958=CARTESIAN_POINT('Ctrl Pts',(16.3594593527494,-17.3694742191139,
-16.956830677183));
#121959=CARTESIAN_POINT('Ctrl Pts',(18.7793599259594,-16.0987959046484,
-17.0840064838644));
#121960=CARTESIAN_POINT('Ctrl Pts',(21.1576455824562,-17.4457552578498,
-17.2111822905458));
#121961=CARTESIAN_POINT('Ctrl Pts',(21.3123868454594,-20.1746006738818,
-17.3383580972273));
#121962=CARTESIAN_POINT('Ctrl Pts',(19.1016182104896,-21.7817858547834,
-17.4655339039087));
#121963=CARTESIAN_POINT('Ctrl Pts',(16.5535826843549,-20.7928181502387,
-17.5927097105901));
#121964=CARTESIAN_POINT('Ctrl Pts',(16.0059447133635,-18.1150140469113,
-17.7198855172716));
#121965=CARTESIAN_POINT('Ctrl Pts',(17.9611281456538,-16.2050926063331,
-17.847061323953));
#121966=CARTESIAN_POINT('Ctrl Pts',(20.6253735344697,-16.8152882071486,
-17.9742371306345));
#121967=CARTESIAN_POINT('Ctrl Pts',(21.55440109729,-19.3857842586047,-18.1014129373159));
#121968=CARTESIAN_POINT('Ctrl Pts',(19.8958857071821,-21.5583101764979,
-18.2285887439973));
#121969=CARTESIAN_POINT('Ctrl Pts',(17.171412295493,-21.3397082732704,-18.3557645506787));
#121970=CARTESIAN_POINT('Ctrl Pts',(15.8805161175613,-18.9305322272779,
-18.4829403573602));
#121971=CARTESIAN_POINT('Ctrl Pts',(17.2075142945774,-16.54105153018,-18.6101161640416));
#121972=CARTESIAN_POINT('Ctrl Pts',(19.9349683619421,-16.3634664140689,
-18.7372919707231));
#121973=CARTESIAN_POINT('Ctrl Pts',(21.5606084977061,-18.5607002000248,
-18.8644677774045));
#121974=CARTESIAN_POINT('Ctrl Pts',(20.5930107759761,-21.1169272666383,
-18.9916435840859));
#121975=CARTESIAN_POINT('Ctrl Pts',(17.9198860504282,-21.6869679347534,
-19.1188193907673));
#121976=CARTESIAN_POINT('Ctrl Pts',(15.9936603441588,-19.7478452776443,
-19.2459951974488));
#121977=CARTESIAN_POINT('Ctrl Pts',(16.5815261871606,-17.078583966977,-19.3731710041302));
#121978=CARTESIAN_POINT('Ctrl Pts',(19.1441531564327,-16.1280656028778,
-19.5003468108116));
#121979=CARTESIAN_POINT('Ctrl Pts',(21.3304900605322,-17.768331748829,-19.6275226174931));
#121980=CARTESIAN_POINT('Ctrl Pts',(21.1347084926027,-20.4945400989296,
-19.7546984241745));
#121981=CARTESIAN_POINT('Ctrl Pts',(18.7364258833193,-21.8055635519036,
-19.881874230856));
#121982=CARTESIAN_POINT('Ctrl Pts',(16.335917684683,-20.4986197454331,-20.0090500375374));
#121983=CARTESIAN_POINT('Ctrl Pts',(16.13550115311,-17.7727479556429,-20.1362258442188));
#121984=CARTESIAN_POINT('Ctrl Pts',(18.3190460623333,-16.1287674194462,
-20.2634016509003));
#121985=CARTESIAN_POINT('Ctrl Pts',(20.8832853969895,-17.0749262060105,
-20.3905774575817));
#121986=CARTESIAN_POINT('Ctrl Pts',(21.4756888902747,-19.7431862770776,
-20.5177532642631));
#121987=CARTESIAN_POINT('Ctrl Pts',(19.5527627818701,-21.6855770682093,
-20.6449290709446));
#121988=CARTESIAN_POINT('Ctrl Pts',(16.8786730502231,-21.1200901556103,
-20.772104877626));
#121989=CARTESIAN_POINT('Ctrl Pts',(15.9067298484541,-18.5654966090028,
-20.8992806843074));
#121990=CARTESIAN_POINT('Ctrl Pts',(17.5286330567039,-16.3655315522399,
-21.0264564909889));
#121991=CARTESIAN_POINT('Ctrl Pts',(20.256382680945,-16.5384221250544,-21.1536322976703));
#121992=CARTESIAN_POINT('Ctrl Pts',(21.5874463526494,-18.9257528612692,
-21.2808081043517));
#121993=CARTESIAN_POINT('Ctrl Pts',(20.3006391779602,-21.3369088308205,
-21.4079839110332));
#121994=CARTESIAN_POINT('Ctrl Pts',(17.5765588536269,-21.5605501870015,
-21.5351597177146));
#121995=CARTESIAN_POINT('Ctrl Pts',(15.9143182549829,-19.3900617201843,
-21.6623355243961));
#121996=CARTESIAN_POINT('Ctrl Pts',(16.8390400444023,-16.8195068044844,
-21.7895113310775));
#121997=CARTESIAN_POINT('Ctrl Pts',(19.5021076033005,-16.2018289998698,
-21.9166871377589));
#121998=CARTESIAN_POINT('Ctrl Pts',(21.4611728203329,-18.1146776111084,
-22.0438816020413));
#121999=CARTESIAN_POINT('Ctrl Pts',(21.0977299961801,-19.8915948627883,
-22.1286841307634));
#122000=CARTESIAN_POINT('Ctrl Pts',(20.5799309501441,-20.506446466246,-22.171094723925));
#122001=CARTESIAN_POINT('Ctrl Pts',(18.1489776385292,-21.138301703768,0.171345817110153));
#122002=CARTESIAN_POINT('Ctrl Pts',(17.4210583610835,-20.9435211508747,
0.128953881549675));
#122003=CARTESIAN_POINT('Ctrl Pts',(16.1877699881095,-19.77288952068,0.0441700104287191));
#122004=CARTESIAN_POINT('Ctrl Pts',(16.6662106246443,-17.2504067355124,
-0.083005796252715));
#122005=CARTESIAN_POINT('Ctrl Pts',(19.0452436391262,-16.2947305011482,
-0.210181602934149));
#122006=CARTESIAN_POINT('Ctrl Pts',(21.1369461776993,-17.7741154785761,
-0.337357409615584));
#122007=CARTESIAN_POINT('Ctrl Pts',(21.0250156451928,-20.3355843150782,
-0.464533216297019));
#122008=CARTESIAN_POINT('Ctrl Pts',(18.8107430711202,-21.6269506071526,
-0.591709022978452));
#122009=CARTESIAN_POINT('Ctrl Pts',(16.5263111681857,-20.4646046776889,
-0.718884829659889));
#122010=CARTESIAN_POINT('Ctrl Pts',(16.2671682231216,-17.9143360270367,
-0.84606063634132));
#122011=CARTESIAN_POINT('Ctrl Pts',(18.2712570171198,-16.3161643914318,
-0.973236443022757));
#122012=CARTESIAN_POINT('Ctrl Pts',(20.6998491681173,-17.1361539837924,
-1.10041224970419));
#122013=CARTESIAN_POINT('Ctrl Pts',(21.3249146812175,-19.6220977928601,
-1.22758805638563));
#122014=CARTESIAN_POINT('Ctrl Pts',(19.5729674648886,-21.4932538336279,
-1.35476386306706));
#122015=CARTESIAN_POINT('Ctrl Pts',(17.0513245079943,-21.0329748042223,
-1.4819396697485));
#122016=CARTESIAN_POINT('Ctrl Pts',(16.0734293667079,-18.6635266109603,
-1.60911547642993));
#122017=CARTESIAN_POINT('Ctrl Pts',(17.5364439501815,-16.5587368924863,
-1.73629128311137));
#122018=CARTESIAN_POINT('Ctrl Pts',(20.0981412048233,-16.6496164712725,
-1.8634670897928));
#122019=CARTESIAN_POINT('Ctrl Pts',(21.4083239228994,-18.852790586328,-1.99064289647423));
#122020=CARTESIAN_POINT('Ctrl Pts',(20.264980246985,-21.1469828950223,-2.11781870315567));
#122021=CARTESIAN_POINT('Ctrl Pts',(17.717057312254,-21.4274147818336,-2.2449945098371));
#122022=CARTESIAN_POINT('Ctrl Pts',(16.1021161259398,-19.4368071709258,
-2.37217031651854));
#122023=CARTESIAN_POINT('Ctrl Pts',(16.9017650663717,-17.0014191111546,
-2.49934612319997));
#122024=CARTESIAN_POINT('Ctrl Pts',(19.3823758238848,-16.3555679294722,
-2.62652192988141));
#122025=CARTESIAN_POINT('Ctrl Pts',(21.2681420125742,-18.0917820305039,
-2.75369773656284));
#122026=CARTESIAN_POINT('Ctrl Pts',(20.8289901877649,-20.6171927218193,
-2.88087354324428));
#122027=CARTESIAN_POINT('Ctrl Pts',(18.467814897281,-21.6148924472776,-3.0080493499257));
#122028=CARTESIAN_POINT('Ctrl Pts',(16.3508479162742,-20.1695536286012,
-3.13522515660715));
#122029=CARTESIAN_POINT('Ctrl Pts',(16.4202750574822,-17.6071849263638,
-3.26240096328857));
#122030=CARTESIAN_POINT('Ctrl Pts',(18.612401227227,-16.278600585146,-3.38957676997001));
#122031=CARTESIAN_POINT('Ctrl Pts',(20.9160867238537,-17.4026942773856,
-3.51675257665145));
#122032=CARTESIAN_POINT('Ctrl Pts',(21.2178430868515,-19.9481798092568,
-3.64392838333288));
#122033=CARTESIAN_POINT('Ctrl Pts',(19.2408275823876,-21.5797321960836,
-3.77110419001432));
#122034=CARTESIAN_POINT('Ctrl Pts',(16.7988292283319,-20.8005033884281,
-3.89827999669575));
#122035=CARTESIAN_POINT('Ctrl Pts',(16.1322299470473,-18.3253874529646,
-4.02545580337718));
#122036=CARTESIAN_POINT('Ctrl Pts',(17.8525932052803,-16.4251496374373,
-4.15263161005862));
#122037=CARTESIAN_POINT('Ctrl Pts',(20.3815924913958,-16.8431401955444,
-4.27980741674006));
#122038=CARTESIAN_POINT('Ctrl Pts',(21.3990279277772,-19.1958787336361,
-4.40698322342148));
#122039=CARTESIAN_POINT('Ctrl Pts',(19.9714656507117,-21.3248736704392,
-4.53415903010293));
#122040=CARTESIAN_POINT('Ctrl Pts',(17.4086054448983,-21.2769042917635,
-4.66133483678435));
#122041=CARTESIAN_POINT('Ctrl Pts',(16.0617124801271,-19.0959795252294,
-4.78851064346579));
#122042=CARTESIAN_POINT('Ctrl Pts',(17.1664774539701,-16.7829624806744,
-4.91568645014722));
#122043=CARTESIAN_POINT('Ctrl Pts',(19.709347072374,-16.4599027344493,-5.04286225682866));
#122044=CARTESIAN_POINT('Ctrl Pts',(21.3573962887413,-18.4231875523662,
-5.1700380635101));
#122045=CARTESIAN_POINT('Ctrl Pts',(20.5986422365255,-20.8716249691852,
-5.29721387019152));
#122046=CARTESIAN_POINT('Ctrl Pts',(18.1291946650469,-21.5589256221392,
-5.42438967687296));
#122047=CARTESIAN_POINT('Ctrl Pts',(16.2146184499352,-19.8545338208328,
-5.55156548355439));
#122048=CARTESIAN_POINT('Ctrl Pts',(16.6114184365535,-17.3221232564787,
-5.67874129023583));
#122049=CARTESIAN_POINT('Ctrl Pts',(18.9555552653643,-16.2850234427458,
-5.80591709691726));
#122050=CARTESIAN_POINT('Ctrl Pts',(21.096428889474,-17.69470908906,-5.9330929035987));
#122051=CARTESIAN_POINT('Ctrl Pts',(21.0699206363647,-20.2578811098868,
-6.06026871028013));
#122052=CARTESIAN_POINT('Ctrl Pts',(18.9003501829765,-21.6229882645151,
-6.18744451696157));
#122053=CARTESIAN_POINT('Ctrl Pts',(16.5781637615641,-20.537629466679,-6.31462032364299));
#122054=CARTESIAN_POINT('Ctrl Pts',(16.2338232826291,-17.9975540484287,
-6.44179613032444));
#122055=CARTESIAN_POINT('Ctrl Pts',(18.1832397634138,-16.3331235511484,
-6.56897193700587));
#122056=CARTESIAN_POINT('Ctrl Pts',(20.6379445772308,-17.0713496498852,
-6.69614774368731));
#122057=CARTESIAN_POINT('Ctrl Pts',(21.3458984135663,-19.5349557185273,
-6.82332355036874));
#122058=CARTESIAN_POINT('Ctrl Pts',(19.6575975681531,-21.4637360977331,
-6.95049935705017));
#122059=CARTESIAN_POINT('Ctrl Pts',(17.1219532788895,-21.0881545031928,
-7.07767516373161));
#122060=CARTESIAN_POINT('Ctrl Pts',(16.0652618013412,-18.7527837366743,
-7.20485097041304));
#122061=CARTESIAN_POINT('Ctrl Pts',(17.4569719804889,-16.6001815270014,
-7.33202677709449));
#122062=CARTESIAN_POINT('Ctrl Pts',(20.0202761062402,-16.6052267959878,
-7.4592025837759));
#122063=CARTESIAN_POINT('Ctrl Pts',(21.4035017398149,-18.7632908224833,
-7.58637839045736));
#122064=CARTESIAN_POINT('Ctrl Pts',(20.3376252150736,-21.094483806738,-7.71355419713877));
#122065=CARTESIAN_POINT('Ctrl Pts',(17.8005220877082,-21.4600808758526,
-7.84073000382022));
#122066=CARTESIAN_POINT('Ctrl Pts',(16.1198270066971,-19.5246694104279,
-7.96790581050164));
#122067=CARTESIAN_POINT('Ctrl Pts',(16.8374733931665,-17.0638693048078,
-8.09508161718309));
#122068=CARTESIAN_POINT('Ctrl Pts',(19.295065229689,-16.335311921419,-8.22225742386451));
#122069=CARTESIAN_POINT('Ctrl Pts',(21.2379145416073,-18.0074034401497,
-8.34943323054596));
#122070=CARTESIAN_POINT('Ctrl Pts',(20.8835776720644,-20.5461036742685,
-8.47660903722738));
#122071=CARTESIAN_POINT('Ctrl Pts',(18.5571367062394,-21.6223127284784,
-8.60378484390882));
#122072=CARTESIAN_POINT('Ctrl Pts',(16.3929568350657,-20.2486755926092,
-8.73096065059025));
#122073=CARTESIAN_POINT('Ctrl Pts',(16.3765387661935,-17.6854190812848,
-8.85813645727169));
#122074=CARTESIAN_POINT('Ctrl Pts',(18.5229450587927,-16.2841719500039,
-8.98531226395313));
#122075=CARTESIAN_POINT('Ctrl Pts',(20.8629811604026,-17.3304914705113,
-9.11248807063455));
#122076=CARTESIAN_POINT('Ctrl Pts',(21.2498091868164,-19.8644444246549,
-9.23966387731599));
#122077=CARTESIAN_POINT('Ctrl Pts',(19.3285384330547,-21.5612862518657,
-9.36683968399743));
#122078=CARTESIAN_POINT('Ctrl Pts',(16.861815568182,-20.864269893559,-9.49401549067886));
#122079=CARTESIAN_POINT('Ctrl Pts',(16.1127057186315,-18.4128645967674,
-9.6211912973603));
#122080=CARTESIAN_POINT('Ctrl Pts',(17.7684706763648,-16.4560825699245,
-9.74836710404172));
#122081=CARTESIAN_POINT('Ctrl Pts',(20.310048861025,-16.7891498710692,-9.87554291072316));
#122082=CARTESIAN_POINT('Ctrl Pts',(21.4057000363191,-19.1064979238893,
-10.0027187174046));
#122083=CARTESIAN_POINT('Ctrl Pts',(20.0502322526962,-21.2821037207635,
-10.129894524086));
#122084=CARTESIAN_POINT('Ctrl Pts',(17.4872030718116,-21.3199839763846,
-10.2570703307675));
#122085=CARTESIAN_POINT('Ctrl Pts',(16.068032687595,-19.1853859073339,-10.3842461374489));
#122086=CARTESIAN_POINT('Ctrl Pts',(17.0947218439171,-16.8366707538674,
-10.5114219441303));
#122087=CARTESIAN_POINT('Ctrl Pts',(19.6253469633683,-16.4286388915877,
-10.6385977508117));
#122088=CARTESIAN_POINT('Ctrl Pts',(21.3382165671608,-18.3356342288226,
-10.7657735574932));
#122089=CARTESIAN_POINT('Ctrl Pts',(20.6618791064926,-20.8081069051386,
-10.8929493641746));
#122090=CARTESIAN_POINT('Ctrl Pts',(18.2168322232895,-21.577716698977,-11.0201251708561));
#122091=CARTESIAN_POINT('Ctrl Pts',(16.2462546761661,-19.9383943918618,
-11.1473009775375));
#122092=CARTESIAN_POINT('Ctrl Pts',(16.5580290567716,-17.3941164527542,
-11.2744767842189));
#122093=CARTESIAN_POINT('Ctrl Pts',(18.8661217218008,-16.2790999750865,
-11.4016525909004));
#122094=CARTESIAN_POINT('Ctrl Pts',(21.0530009074768,-17.6163033713916,
-11.5288283975818));
#122095=CARTESIAN_POINT('Ctrl Pts',(21.1123406939717,-20.1789255217625,
-11.6560042042632));
#122096=CARTESIAN_POINT('Ctrl Pts',(18.989700510219,-21.6159196575024,-11.7831800109447));
#122097=CARTESIAN_POINT('Ctrl Pts',(16.6324709789039,-20.6089328489849,
-11.9103558176261));
#122098=CARTESIAN_POINT('Ctrl Pts',(16.203263888843,-18.0818129923747,-12.0375316243075));
#122099=CARTESIAN_POINT('Ctrl Pts',(18.0958501055707,-16.3530357053638,
-12.164707430989));
#122100=CARTESIAN_POINT('Ctrl Pts',(20.5738992423879,-17.0086468487652,
-12.2918832376704));
#122101=CARTESIAN_POINT('Ctrl Pts',(21.3639550213402,-19.4471638903247,
-12.4190590443519));
#122102=CARTESIAN_POINT('Ctrl Pts',(19.7411903016307,-21.4313987958485,
-12.5462348510332));
#122103=CARTESIAN_POINT('Ctrl Pts',(17.1943909934554,-21.140939195026,-12.6734106577147));
#122104=CARTESIAN_POINT('Ctrl Pts',(16.0600873898727,-18.8422637436558,
-12.8005864643961));
#122105=CARTESIAN_POINT('Ctrl Pts',(17.3789326443482,-16.6442644964813,
-12.9277622710776));
#122106=CARTESIAN_POINT('Ctrl Pts',(19.9409680926688,-16.563469339566,-13.054938077759));
#122107=CARTESIAN_POINT('Ctrl Pts',(21.3956852288542,-18.6740028146668,
-13.1821138844404));
#122108=CARTESIAN_POINT('Ctrl Pts',(20.4084713703825,-21.0395814528595,
-13.3092896911219));
#122109=CARTESIAN_POINT('Ctrl Pts',(17.8850339589992,-21.4899336779714,
-13.4364654978033));
#122110=CARTESIAN_POINT('Ctrl Pts',(16.1404701974589,-19.6118892754737,
-13.5636413044848));
#122111=CARTESIAN_POINT('Ctrl Pts',(16.7753090571362,-17.1284374200765,
-13.6908171111662));
#122112=CARTESIAN_POINT('Ctrl Pts',(19.2071252868205,-16.3179910487006,
-13.8179929178476));
#122113=CARTESIAN_POINT('Ctrl Pts',(21.2048784313142,-17.9240844051089,
-13.945168724529));
#122114=CARTESIAN_POINT('Ctrl Pts',(20.9357539750881,-20.4732265201925,
-14.0723445312105));
#122115=CARTESIAN_POINT('Ctrl Pts',(18.6466569029825,-21.6267377209658,
-14.1995203378919));
#122116=CARTESIAN_POINT('Ctrl Pts',(16.4376917012663,-20.3263430756987,
-14.3266961445733));
#122117=CARTESIAN_POINT('Ctrl Pts',(16.3354468386715,-17.7650739598295,
-14.4538719512548));
#122118=CARTESIAN_POINT('Ctrl Pts',(18.4337256305968,-16.2927358168784,
-14.5810477579362));
#122119=CARTESIAN_POINT('Ctrl Pts',(20.8074875193202,-17.2601075093917,
-14.7082235646177));
#122120=CARTESIAN_POINT('Ctrl Pts',(21.2789533042171,-19.7796855513471,
-14.8353993712991));
#122121=CARTESIAN_POINT('Ctrl Pts',(19.4155823901109,-21.5399134719006,
-14.9625751779805));
#122122=CARTESIAN_POINT('Ctrl Pts',(16.9269019368522,-20.9258914060103,
-15.089750984662));
#122123=CARTESIAN_POINT('Ctrl Pts',(16.0961217953763,-18.5009464886232,
-15.2169267913434));
#122124=CARTESIAN_POINT('Ctrl Pts',(17.6854311814566,-16.489815172386,-15.3441025980248));
#122125=CARTESIAN_POINT('Ctrl Pts',(20.2367373770296,-16.7375856150594,
-15.4712784047062));
#122126=CARTESIAN_POINT('Ctrl Pts',(21.4093752995786,-19.0169438138584,
-15.5984542113877));
#122127=CARTESIAN_POINT('Ctrl Pts',(20.1275224372825,-21.2367200943101,
-15.7256300180691));
#122128=CARTESIAN_POINT('Ctrl Pts',(17.5671992305365,-21.3604074939539,
-15.8528058247506));
#122129=CARTESIAN_POINT('Ctrl Pts',(16.0773433099501,-19.2745305005226,
-15.979981631432));
#122130=CARTESIAN_POINT('Ctrl Pts',(17.0248050117741,-16.8927517913624,
-16.1071574381134));
#122131=CARTESIAN_POINT('Ctrl Pts',(19.5403470306901,-16.4002055022689,
-16.2343332447949));
#122132=CARTESIAN_POINT('Ctrl Pts',(21.3161156964891,-18.2487722826149,
-16.3615090514763));
#122133=CARTESIAN_POINT('Ctrl Pts',(20.7229534749337,-20.7425068464271,
-16.4886848581577));
#122134=CARTESIAN_POINT('Ctrl Pts',(18.3050498885018,-21.5935625100306,
-16.6158606648392));
#122135=CARTESIAN_POINT('Ctrl Pts',(16.2806814057228,-20.021148524541,-16.7430364715206));
#122136=CARTESIAN_POINT('Ctrl Pts',(16.5070804630683,-17.4678571266262,
-16.870212278202));
#122137=CARTESIAN_POINT('Ctrl Pts',(18.776539977334,-16.2761746987364,-16.9973880848835));
#122138=CARTESIAN_POINT('Ctrl Pts',(21.0069717027245,-17.5393959043074,
-17.1245638915649));
#122139=CARTESIAN_POINT('Ctrl Pts',(21.1520929673995,-20.0985936915781,
-17.2517396982463));
#122140=CARTESIAN_POINT('Ctrl Pts',(19.0787640182614,-21.6058629324566,
-17.3789155049278));
#122141=CARTESIAN_POINT('Ctrl Pts',(16.6891354808367,-20.6783776501158,
-17.5060913116092));
#122142=CARTESIAN_POINT('Ctrl Pts',(16.1755432211384,-18.1670480248764,
-17.6332671182907));
#122143=CARTESIAN_POINT('Ctrl Pts',(18.0091762603091,-16.3758631171963,
-17.760442924972));
#122144=CARTESIAN_POINT('Ctrl Pts',(20.5077900930114,-16.9481239064058,
-17.8876187316535));
#122145=CARTESIAN_POINT('Ctrl Pts',(21.3790616092047,-19.3588166369015,
-18.0147945383349));
#122146=CARTESIAN_POINT('Ctrl Pts',(19.8236532699919,-21.3962803529462,
-18.1419703450164));
#122147=CARTESIAN_POINT('Ctrl Pts',(17.2685556870694,-21.1912685542763,
-18.2691461516978));
#122148=CARTESIAN_POINT('Ctrl Pts',(16.0579123055315,-18.931866841806,-18.3963219583793));
#122149=CARTESIAN_POINT('Ctrl Pts',(17.3024132869284,-16.6909360522447,
-18.5234977650607));
#122150=CARTESIAN_POINT('Ctrl Pts',(19.8603062232868,-16.5243910975421,
-18.6506735717421));
#122151=CARTESIAN_POINT('Ctrl Pts',(21.3848831062071,-18.5850266359637,
-18.7778493784235));
#122152=CARTESIAN_POINT('Ctrl Pts',(20.4774392715833,-20.9823374598767,
-18.905025185105));
#122153=CARTESIAN_POINT('Ctrl Pts',(17.9704981152505,-21.5169396795275,
-19.0322009917864));
#122154=CARTESIAN_POINT('Ctrl Pts',(16.164022550051,-19.6983689447528,-19.1593767984678));
#122155=CARTESIAN_POINT('Ctrl Pts',(16.7153417841063,-17.1950510214384,
-19.2865526051493));
#122156=CARTESIAN_POINT('Ctrl Pts',(19.1186546397307,-16.3036247501402,
-19.4137284118307));
#122157=CARTESIAN_POINT('Ctrl Pts',(21.1690707367099,-17.8419183693358,
-19.5409042185122));
#122158=CARTESIAN_POINT('Ctrl Pts',(20.9854605723195,-20.3986430325311,
-19.6680800251936));
#122159=CARTESIAN_POINT('Ctrl Pts',(18.7362750703233,-21.6281624110196,
-19.795255831875));
#122160=CARTESIAN_POINT('Ctrl Pts',(16.4850023400387,-20.4024690544242,
-19.9224316385565));
#122161=CARTESIAN_POINT('Ctrl Pts',(16.2970453597273,-17.8460600281632,
-20.0496074452379));
#122162=CARTESIAN_POINT('Ctrl Pts',(18.3448430353522,-16.3042829359788,
-20.1767832519193));
#122163=CARTESIAN_POINT('Ctrl Pts',(20.7496680183763,-17.1916206571837,
-20.3039590586007));
#122164=CARTESIAN_POINT('Ctrl Pts',(21.305242804797,-19.6939995862426,-20.4311348652822));
#122165=CARTESIAN_POINT('Ctrl Pts',(19.5018617071349,-21.5156352807657,
-20.5583106719636));
#122166=CARTESIAN_POINT('Ctrl Pts',(16.9940155374735,-20.9853037174782,
-20.6854864786451));
#122167=CARTESIAN_POINT('Ctrl Pts',(16.082496373835,-18.5895248604405,-20.8126622853265));
#122168=CARTESIAN_POINT('Ctrl Pts',(17.6035686476012,-16.5263278496229,
-20.9398380920079));
#122169=CARTESIAN_POINT('Ctrl Pts',(20.1617387665729,-16.6884701127161,
-21.0670138986894));
#122170=CARTESIAN_POINT('Ctrl Pts',(21.4100524978415,-18.9273846007665,
-21.1941897053708));
#122171=CARTESIAN_POINT('Ctrl Pts',(20.2032439132434,-21.1886431483515,
-21.3213655120522));
#122172=CARTESIAN_POINT('Ctrl Pts',(17.6485149801115,-21.3983811058473,
-21.4485413187337));
#122173=CARTESIAN_POINT('Ctrl Pts',(16.0896130221739,-19.3628281760474,
-21.5757171254151));
#122174=CARTESIAN_POINT('Ctrl Pts',(16.9568464474972,-16.9520802407969,
-21.7028929320966));
#122175=CARTESIAN_POINT('Ctrl Pts',(19.4543556739431,-16.3728024035369,
-21.8300687387779));
#122176=CARTESIAN_POINT('Ctrl Pts',(21.291629173971,-18.1667325047092,-21.9572632030605));
#122177=CARTESIAN_POINT('Ctrl Pts',(20.9507809654552,-19.8331818652868,
-22.0420657317825));
#122178=CARTESIAN_POINT('Ctrl Pts',(20.4651725960397,-20.4098092014579,
-22.084476324944));
#122179=CARTESIAN_POINT('Ctrl Pts',(18.187758406819,-20.9933731243335,0.257964216091064));
#122180=CARTESIAN_POINT('Ctrl Pts',(17.5080924453001,-20.811504453082,0.215572280530586));
#122181=CARTESIAN_POINT('Ctrl Pts',(16.3565579911106,-19.7184732651834,
0.13078840940963));
#122182=CARTESIAN_POINT('Ctrl Pts',(16.8032830955771,-17.3632042941351,
0.00361260272819585));
#122183=CARTESIAN_POINT('Ctrl Pts',(19.0246114919716,-16.4708792426415,
-0.123563203953239));
#122184=CARTESIAN_POINT('Ctrl Pts',(20.9776563709031,-17.8521967105185,
-0.250739010634673));
#122185=CARTESIAN_POINT('Ctrl Pts',(20.8731456437434,-20.2438673718189,
-0.377914817316107));
#122186=CARTESIAN_POINT('Ctrl Pts',(18.805655820692,-21.4496297959928,-0.505090623997542));
#122187=CARTESIAN_POINT('Ctrl Pts',(16.6726574870295,-20.3643350548799,
-0.632266430678976));
#122188=CARTESIAN_POINT('Ctrl Pts',(16.4306929665323,-17.9831221260791,
-0.75944223736041));
#122189=CARTESIAN_POINT('Ctrl Pts',(18.3019319614957,-16.490892293676,-0.886618044041845));
#122190=CARTESIAN_POINT('Ctrl Pts',(20.5695342500862,-17.2565252862285,
-1.01379385072328));
#122191=CARTESIAN_POINT('Ctrl Pts',(21.1531645592934,-19.5776774271649,
-1.14096965740471));
#122192=CARTESIAN_POINT('Ctrl Pts',(19.5173528337202,-21.3247956983873,
-1.26814546408615));
#122193=CARTESIAN_POINT('Ctrl Pts',(17.1628680192514,-20.8950282794151,
-1.39532127076758));
#122194=CARTESIAN_POINT('Ctrl Pts',(16.249796938349,-18.6826493324063,-1.52249707744901));
#122195=CARTESIAN_POINT('Ctrl Pts',(17.6158291954999,-16.7173848145856,
-1.64967288413045));
#122196=CARTESIAN_POINT('Ctrl Pts',(20.0077131332437,-16.8022400426472,
-1.77684869081188));
#122197=CARTESIAN_POINT('Ctrl Pts',(21.2310446542488,-18.8593671166236,
-1.90402449749332));
#122198=CARTESIAN_POINT('Ctrl Pts',(20.1634925191223,-21.0014788448218,
-2.03120030417475));
#122199=CARTESIAN_POINT('Ctrl Pts',(17.784469810194,-21.2633210763656,-2.15837611085619));
#122200=CARTESIAN_POINT('Ctrl Pts',(16.2765820701628,-19.4046696052546,
-2.28555191753762));
#122201=CARTESIAN_POINT('Ctrl Pts',(17.0232227799449,-17.1307219044541,
-2.41272772421906));
#122202=CARTESIAN_POINT('Ctrl Pts',(19.3393953939956,-16.5276837957002,
-2.53990353090049));
#122203=CARTESIAN_POINT('Ctrl Pts',(21.1001553155256,-18.148805344399,-2.66707933758192));
#122204=CARTESIAN_POINT('Ctrl Pts',(20.6901145919042,-20.5068081325184,
-2.79425514426337));
#122205=CARTESIAN_POINT('Ctrl Pts',(18.4854601420967,-21.4383709640324,
-2.92143095094479));
#122206=CARTESIAN_POINT('Ctrl Pts',(16.5088255848986,-20.0888427562296,
-3.04860675762623));
#122207=CARTESIAN_POINT('Ctrl Pts',(16.5736504441196,-17.6963318807336,
-3.17578256430766));
#122208=CARTESIAN_POINT('Ctrl Pts',(18.6204619342047,-16.4558185687336,
-3.3029583709891));
#122209=CARTESIAN_POINT('Ctrl Pts',(20.7714375528147,-17.5053967896241,
-3.43013417767053));
#122210=CARTESIAN_POINT('Ctrl Pts',(21.0531906742887,-19.8821436696115,
-3.55730998435197));
#122211=CARTESIAN_POINT('Ctrl Pts',(19.2072302973436,-21.4055414640101,
-3.6844857910334));
#122212=CARTESIAN_POINT('Ctrl Pts',(16.9271104945531,-20.6779672491097,
-3.81166159771483));
#122213=CARTESIAN_POINT('Ctrl Pts',(16.3046996648085,-18.3669252087745,
-3.93883740439627));
#122214=CARTESIAN_POINT('Ctrl Pts',(17.9110211132137,-16.5926529755442,
-4.0660132110777));
#122215=CARTESIAN_POINT('Ctrl Pts',(20.2723746104174,-16.9829351996645,
-4.19318901775914));
#122216=CARTESIAN_POINT('Ctrl Pts',(21.2223648848585,-19.179712164146,-4.32036482444056));
#122217=CARTESIAN_POINT('Ctrl Pts',(19.8894348227856,-21.1675773514354,
-4.44754063112201));
#122218=CARTESIAN_POINT('Ctrl Pts',(17.4964650251793,-21.1227878330214,
-4.57471643780344));
#122219=CARTESIAN_POINT('Ctrl Pts',(16.2388567568882,-19.0864352120986,
-4.70189224448488));
#122220=CARTESIAN_POINT('Ctrl Pts',(17.2703875480967,-16.9267466280655,
-4.8290680511663));
#122221=CARTESIAN_POINT('Ctrl Pts',(19.6446919218926,-16.6251023113816,
-4.95624385784775));
#122222=CARTESIAN_POINT('Ctrl Pts',(21.1834929812674,-18.4582422004466,
-5.08341966452918));
#122223=CARTESIAN_POINT('Ctrl Pts',(20.4750362630098,-20.7443742245365,
-5.21059547121061));
#122224=CARTESIAN_POINT('Ctrl Pts',(18.1692868343382,-21.386114144905,-5.33777127789205));
#122225=CARTESIAN_POINT('Ctrl Pts',(16.3816266851093,-19.7947054154853,
-5.46494708457348));
#122226=CARTESIAN_POINT('Ctrl Pts',(16.7521230475383,-17.4301667715549,
-5.59212289125491));
#122227=CARTESIAN_POINT('Ctrl Pts',(18.9408685046945,-16.4618156591,-5.71929869793635));
#122228=CARTESIAN_POINT('Ctrl Pts',(20.9398249485008,-17.7780541211498,
-5.84647450461778));
#122229=CARTESIAN_POINT('Ctrl Pts',(20.9150739109944,-20.1713150637459,
-5.97365031129922));
#122230=CARTESIAN_POINT('Ctrl Pts',(18.8893229328647,-21.4459301145832,
-6.10082611798065));
#122231=CARTESIAN_POINT('Ctrl Pts',(16.7210728042601,-20.4325190760503,
-6.22800192466209));
#122232=CARTESIAN_POINT('Ctrl Pts',(16.3995584413949,-18.0608236766186,
-6.35517773134351));
#122233=CARTESIAN_POINT('Ctrl Pts',(18.2197493167659,-16.5067272412486,
-6.48235353802496));
#122234=CARTESIAN_POINT('Ctrl Pts',(20.5117332760072,-17.1960167912891,
-6.60952934470639));
#122235=CARTESIAN_POINT('Ctrl Pts',(21.1727572930827,-19.4963119467122,
-6.73670515138783));
#122236=CARTESIAN_POINT('Ctrl Pts',(19.5963728601034,-21.2972346748364,
-6.86388095806926));
#122237=CARTESIAN_POINT('Ctrl Pts',(17.2288148528754,-20.9465501504785,
-6.99105676475069));
#122238=CARTESIAN_POINT('Ctrl Pts',(16.2421707958078,-18.7659896588004,
-7.11823257143212));
#122239=CARTESIAN_POINT('Ctrl Pts',(17.5416253732237,-16.7560821100692,
-7.24540837811357));
#122240=CARTESIAN_POINT('Ctrl Pts',(19.935009663591,-16.7607929313141,-7.37258418479499));
#122241=CARTESIAN_POINT('Ctrl Pts',(21.2265421306802,-18.7758002364295,
-7.49975999147643));
#122242=CARTESIAN_POINT('Ctrl Pts',(20.2313218974823,-20.9524598884302,
-7.62693579815786));
#122243=CARTESIAN_POINT('Ctrl Pts',(17.8624017576224,-21.2938217553397,
-7.7541116048393));
#122244=CARTESIAN_POINT('Ctrl Pts',(16.2931189076558,-19.4867075115756,
-7.88128741152073));
#122245=CARTESIAN_POINT('Ctrl Pts',(16.9631929617487,-17.189032313632,-8.00846321820217));
#122246=CARTESIAN_POINT('Ctrl Pts',(19.2578725647568,-16.5087705458158,
-8.1356390248836));
#122247=CARTESIAN_POINT('Ctrl Pts',(21.0719316047989,-18.0700201582916,
-8.26281483156504));
#122248=CARTESIAN_POINT('Ctrl Pts',(20.7410835058385,-20.440431533692,-8.38999063824647));
#122249=CARTESIAN_POINT('Ctrl Pts',(18.5688608639229,-21.4452993594099,
-8.5171664449279));
#122250=CARTESIAN_POINT('Ctrl Pts',(16.5481431296672,-20.1627197744802,
-8.64434225160934));
#122251=CARTESIAN_POINT('Ctrl Pts',(16.5328134043638,-17.7693799422089,
-8.77151805829078));
#122252=CARTESIAN_POINT('Ctrl Pts',(18.5369357595085,-16.461020611282,-8.89869386497221));
#122253=CARTESIAN_POINT('Ctrl Pts',(20.7218523241179,-17.4379802618865,
-9.02586967165363));
#122254=CARTESIAN_POINT('Ctrl Pts',(21.0830377613791,-19.8039590515472,
-9.15304547833508));
#122255=CARTESIAN_POINT('Ctrl Pts',(19.2891268503013,-21.3883182899558,
-9.28022128501651));
#122256=CARTESIAN_POINT('Ctrl Pts',(16.9859215091302,-20.7375067122967,
-9.40739709169795));
#122257=CARTESIAN_POINT('Ctrl Pts',(16.2864696853447,-18.4486035471504,
-9.53457289837939));
#122258=CARTESIAN_POINT('Ctrl Pts',(17.8324750143917,-16.621535383186,-9.6617487050608));
#122259=CARTESIAN_POINT('Ctrl Pts',(20.2055735627832,-16.9325238602014,
-9.78892451174226));
#122260=CARTESIAN_POINT('Ctrl Pts',(21.2285947034771,-19.0962563526568,
-9.91610031842368));
#122261=CARTESIAN_POINT('Ctrl Pts',(19.9629800357399,-21.1276425951086,
-10.0432761251051));
#122262=CARTESIAN_POINT('Ctrl Pts',(17.569852464315,-21.1630117921569,-10.1704519317865));
#122263=CARTESIAN_POINT('Ctrl Pts',(16.2447580017361,-19.1699149007699,
-10.297627738468));
#122264=CARTESIAN_POINT('Ctrl Pts',(17.2033885727816,-16.9768946132505,
-10.4248035451494));
#122265=CARTESIAN_POINT('Ctrl Pts',(19.5662601278407,-16.5959109292081,
-10.5519793518308));
#122266=CARTESIAN_POINT('Ctrl Pts',(21.1655846714952,-18.3764927322373,
-10.6791551585123));
#122267=CARTESIAN_POINT('Ctrl Pts',(20.5340812002182,-20.6850667334291,
-10.8063309651937));
#122268=CARTESIAN_POINT('Ctrl Pts',(18.2511149533807,-21.4036595729525,
-10.9335067718751));
#122269=CARTESIAN_POINT('Ctrl Pts',(16.4111657655901,-19.8730069214463,
-11.0606825785565));
#122270=CARTESIAN_POINT('Ctrl Pts',(16.7022728165186,-17.4973875836496,
-11.187858385238));
#122271=CARTESIAN_POINT('Ctrl Pts',(18.8573634550803,-16.4562848544257,
-11.3150341919194));
#122272=CARTESIAN_POINT('Ctrl Pts',(20.8992757804055,-17.7048458697147,
-11.4422099986009));
#122273=CARTESIAN_POINT('Ctrl Pts',(20.9546819693801,-20.0975933924253,
-11.5693858052823));
#122274=CARTESIAN_POINT('Ctrl Pts',(18.9727502825159,-21.4393300811306,
-11.6965616119637));
#122275=CARTESIAN_POINT('Ctrl Pts',(16.7717800299571,-20.4990958015143,
-11.8237374186452));
#122276=CARTESIAN_POINT('Ctrl Pts',(16.3710248108061,-18.1394971476037,
-11.9509132253266));
#122277=CARTESIAN_POINT('Ctrl Pts',(18.1381526649597,-16.5253194311522,
-12.078089032008));
#122278=CARTESIAN_POINT('Ctrl Pts',(20.4519334665563,-17.137470519836,-12.2052648386895));
#122279=CARTESIAN_POINT('Ctrl Pts',(21.1896169395636,-19.4143397841694,
-12.3324406453709));
#122280=CARTESIAN_POINT('Ctrl Pts',(19.6744242832976,-21.2670409925706,
-12.4596164520523));
#122281=CARTESIAN_POINT('Ctrl Pts',(17.2964507164198,-20.9958357779372,
-12.5867922587338));
#122282=CARTESIAN_POINT('Ctrl Pts',(16.2373393928556,-18.8495380918013,
-12.7139680654152));
#122283=CARTESIAN_POINT('Ctrl Pts',(17.4687592161129,-16.7972428469345,
-12.8411438720966));
#122284=CARTESIAN_POINT('Ctrl Pts',(19.8609589288869,-16.7218035506933,
-12.9683196787781));
#122285=CARTESIAN_POINT('Ctrl Pts',(21.219243771367,-18.6924310750883,-13.0954954854595));
#122286=CARTESIAN_POINT('Ctrl Pts',(20.2974717052425,-20.9011969774254,
-13.222671292141));
#122287=CARTESIAN_POINT('Ctrl Pts',(17.9413113895561,-21.3216956337831,
-13.3498470988224));
#122288=CARTESIAN_POINT('Ctrl Pts',(16.3123936741481,-19.5681456260435,
-13.4770229055038));
#122289=CARTESIAN_POINT('Ctrl Pts',(16.9051494608697,-17.2493202487194,
-13.6041987121852));
#122290=CARTESIAN_POINT('Ctrl Pts',(19.1757621059772,-16.4925978629714,
-13.7313745188667));
#122291=CARTESIAN_POINT('Ctrl Pts',(21.0410854376991,-17.9922242902351,
-13.8585503255481));
#122292=CARTESIAN_POINT('Ctrl Pts',(20.7898010742036,-20.3723853608092,
-13.9857261322295));
#122293=CARTESIAN_POINT('Ctrl Pts',(18.6524468225313,-21.449431021899,-14.112901938911));
#122294=CARTESIAN_POINT('Ctrl Pts',(16.5899125494253,-20.2352387284471,
-14.2400777455924));
#122295=CARTESIAN_POINT('Ctrl Pts',(16.4944454351463,-17.8437545484231,
-14.3672535522739));
#122296=CARTESIAN_POINT('Ctrl Pts',(18.4536306316875,-16.4690167847506,
-14.4944293589553));
#122297=CARTESIAN_POINT('Ctrl Pts',(20.67003732197,-17.3722620097506,-14.6216051656367));
#122298=CARTESIAN_POINT('Ctrl Pts',(21.1102499333731,-19.7248187912068,
-14.7487809723181));
#122299=CARTESIAN_POINT('Ctrl Pts',(19.3704007176106,-21.3683622982746,
-14.8759567789996));
#122300=CARTESIAN_POINT('Ctrl Pts',(17.0466933429237,-20.7950433730338,
-15.003132585681));
#122301=CARTESIAN_POINT('Ctrl Pts',(16.2709851000421,-18.5308465452073,
-15.1303083923625));
#122302=CARTESIAN_POINT('Ctrl Pts',(17.7549401559266,-16.6530318724217,
-15.2574841990439));
#122303=CARTESIAN_POINT('Ctrl Pts',(20.137121851441,-16.8843777666347,-15.3846600057253));
#122304=CARTESIAN_POINT('Ctrl Pts',(21.2320263358222,-19.0126387288515,
-15.5118358124068));
#122305=CARTESIAN_POINT('Ctrl Pts',(20.0351467020866,-21.085267421011,-15.6390116190882));
#122306=CARTESIAN_POINT('Ctrl Pts',(17.6445457274587,-21.2007556599016,
-15.7661874257696));
#122307=CARTESIAN_POINT('Ctrl Pts',(16.2534514287292,-19.2531501543497,
-15.893363232451));
#122308=CARTESIAN_POINT('Ctrl Pts',(17.1381064839328,-17.0292580736685,
-16.0205390391325));
#122309=CARTESIAN_POINT('Ctrl Pts',(19.4868947878054,-16.5693623715735,
-16.1477148458139));
#122310=CARTESIAN_POINT('Ctrl Pts',(21.1449488537871,-18.2953888103906,
-16.2748906524954));
#122311=CARTESIAN_POINT('Ctrl Pts',(20.5911069867814,-20.6238152617876,
-16.4020664591768));
#122312=CARTESIAN_POINT('Ctrl Pts',(18.3334847244627,-21.4184549750521,
-16.5292422658582));
#122313=CARTESIAN_POINT('Ctrl Pts',(16.4433103686679,-19.950275334167,-16.6564180725397));
#122314=CARTESIAN_POINT('Ctrl Pts',(16.6547015733873,-17.5662400341386,
-16.7835938792211));
#122315=CARTESIAN_POINT('Ctrl Pts',(18.7737200287087,-16.4535534928245,
-16.9107696859025));
#122316=CARTESIAN_POINT('Ctrl Pts',(20.8562978229928,-17.633036550765,-17.037945492584));
#122317=CARTESIAN_POINT('Ctrl Pts',(20.9917990893397,-20.0225867092743,
-17.1651212992654));
#122318=CARTESIAN_POINT('Ctrl Pts',(19.0559098260331,-21.4299400101298,
-17.2922971059468));
#122319=CARTESIAN_POINT('Ctrl Pts',(16.8246882773183,-20.563937149993,-17.4194729126283));
#122320=CARTESIAN_POINT('Ctrl Pts',(16.3451417289135,-18.2190820028416,
-17.5466487193097));
#122321=CARTESIAN_POINT('Ctrl Pts',(18.0572243749645,-16.5466336280595,
-17.6738245259911));
#122322=CARTESIAN_POINT('Ctrl Pts',(20.3902066515531,-17.0809596056631,
-17.8010003326726));
#122323=CARTESIAN_POINT('Ctrl Pts',(21.2037221211194,-19.3318490151982,
-17.928176139354));
#122324=CARTESIAN_POINT('Ctrl Pts',(19.7514208328018,-21.2342505293946,
-18.0553519460354));
#122325=CARTESIAN_POINT('Ctrl Pts',(17.3656990786459,-21.0428288352822,
-18.1825277527169));
#122326=CARTESIAN_POINT('Ctrl Pts',(16.2353084935018,-18.9332014563341,
-18.3097035593983));
#122327=CARTESIAN_POINT('Ctrl Pts',(17.3973122792794,-16.8408205743096,
-18.4368793660797));
#122328=CARTESIAN_POINT('Ctrl Pts',(19.7856440846313,-16.6853157810153,
-18.5640551727612));
#122329=CARTESIAN_POINT('Ctrl Pts',(21.2091577147082,-18.6093530719028,
-18.6912309794426));
#122330=CARTESIAN_POINT('Ctrl Pts',(20.3618677671906,-20.8477476531151,
-18.8184067861241));
#122331=CARTESIAN_POINT('Ctrl Pts',(18.0211101800729,-21.3469114243016,
-18.9455825928055));
#122332=CARTESIAN_POINT('Ctrl Pts',(16.3343847559432,-19.6488926118612,
-19.072758399487));
#122333=CARTESIAN_POINT('Ctrl Pts',(16.849157381052,-17.3115180758999,-19.1999342061683));
#122334=CARTESIAN_POINT('Ctrl Pts',(19.0931561230287,-16.4791838974025,
-19.3271100128498));
#122335=CARTESIAN_POINT('Ctrl Pts',(21.0076514128875,-17.9155049898426,
-19.4542858195312));
#122336=CARTESIAN_POINT('Ctrl Pts',(20.8362126520363,-20.3027459661324,
-19.5814616262127));
#122337=CARTESIAN_POINT('Ctrl Pts',(18.7361242573274,-21.4507612701356,
-19.7086374328941));
#122338=CARTESIAN_POINT('Ctrl Pts',(16.6340869953943,-20.3063183634152,
-19.8358132395755));
#122339=CARTESIAN_POINT('Ctrl Pts',(16.4585895663445,-17.9193721006837,
-19.9629890462569));
#122340=CARTESIAN_POINT('Ctrl Pts',(18.3706400083713,-16.4797984525115,
-20.0901648529384));
#122341=CARTESIAN_POINT('Ctrl Pts',(20.6160506397633,-17.3083151083569,
-20.2173406596198));
#122342=CARTESIAN_POINT('Ctrl Pts',(21.1347967193193,-19.6448128954076,
-20.3445164663014));
#122343=CARTESIAN_POINT('Ctrl Pts',(19.4509606323997,-21.3456934933219,
-20.4716922729828));
#122344=CARTESIAN_POINT('Ctrl Pts',(17.1093580247237,-20.8505172793461,
-20.5988680796641));
#122345=CARTESIAN_POINT('Ctrl Pts',(16.2582628992159,-18.6135531118782,
-20.7260438863456));
#122346=CARTESIAN_POINT('Ctrl Pts',(17.6785042384983,-16.6871241470058,
-20.853219693027));
#122347=CARTESIAN_POINT('Ctrl Pts',(20.0670948522008,-16.8385181003778,
-20.9803954997085));
#122348=CARTESIAN_POINT('Ctrl Pts',(21.2326586430337,-18.9290163402638,
-21.1075713063899));
#122349=CARTESIAN_POINT('Ctrl Pts',(20.1058486485267,-21.0403774658824,
-21.2347471130714));
#122350=CARTESIAN_POINT('Ctrl Pts',(17.7204711065961,-21.2362120246932,
-21.3619229197528));
#122351=CARTESIAN_POINT('Ctrl Pts',(16.264907789365,-19.3355946319105,-21.4890987264342));
#122352=CARTESIAN_POINT('Ctrl Pts',(17.0746528505921,-17.0846536771093,
-21.6162745331156));
#122353=CARTESIAN_POINT('Ctrl Pts',(19.4066037445858,-16.543775807204,-21.743450339797));
#122354=CARTESIAN_POINT('Ctrl Pts',(21.1220855276092,-18.2187873983098,
-21.8706448040796));
#122355=CARTESIAN_POINT('Ctrl Pts',(20.8038319347303,-19.7747688677855,
-21.9554473328015));
#122356=CARTESIAN_POINT('Ctrl Pts',(20.3504142419353,-20.3131719366696,
-21.9978579259631));
#122357=CARTESIAN_POINT('Ctrl Pts',(18.0722627314315,-21.4249949024184,
8.33751470641353E-16));
#122358=CARTESIAN_POINT('Ctrl Pts',(17.9903580532758,-21.3953391176122,
-1.14232169905555E-14));
#122359=CARTESIAN_POINT('Ctrl Pts',(17.9103568112513,-21.3612556170403,
-1.32314169705265E-14));
#122360=CARTESIAN_POINT('Ctrl Pts',(17.8324629519401,-21.3230651201994,
1.30451205393456E-15));
#122361=CARTESIAN_POINT('Ctrl Pts',(17.7532833251897,-21.2842442258181,
1.60803807142514E-14));
#122362=CARTESIAN_POINT('Ctrl Pts',(17.6762805476582,-21.2411789324033,
2.98180794711572E-15));
#122363=CARTESIAN_POINT('Ctrl Pts',(17.6016979156742,-21.1941602566503,
-2.64718802434061E-15));
#122364=CARTESIAN_POINT('Ctrl Pts',(17.5268866858286,-21.1469974673358,
-8.29343702652826E-15));
#122365=CARTESIAN_POINT('Ctrl Pts',(17.4545098273189,-21.0958562232523,
8.2392653840351E-15));
#122366=CARTESIAN_POINT('Ctrl Pts',(17.384851733613,-21.0409959626311,1.8547663405144E-14));
#122367=CARTESIAN_POINT('Ctrl Pts',(17.3596729290768,-21.0211660232012,
2.22737650689451E-14));
#122368=CARTESIAN_POINT('Ctrl Pts',(17.3348497590583,-21.0008499098516,
1.90970525389729E-14));
#122369=CARTESIAN_POINT('Ctrl Pts',(17.3103971449292,-20.9800590889455,
1.05887520973624E-14));
#122370=CARTESIAN_POINT('Ctrl Pts',(17.2929747331899,-20.9652456935222,
4.71885765034174E-15));
#122371=CARTESIAN_POINT('Ctrl Pts',(17.2757404518089,-20.9501913039064,
6.92286535120819E-16));
#122372=CARTESIAN_POINT('Ctrl Pts',(17.2586999683651,-20.9348999714627,
1.49116829994966E-14));
#122373=CARTESIAN_POINT('Ctrl Pts',(17.2462568322336,-20.9237340833671,
2.52948324270246E-14));
#122374=CARTESIAN_POINT('Ctrl Pts',(17.2339149535825,-20.9124397717598,
2.54593689853369E-14));
#122375=CARTESIAN_POINT('Ctrl Pts',(17.2216943473019,-20.9010355554554,
1.92762472650543E-14));
#122376=CARTESIAN_POINT('Ctrl Pts',(17.1582585289398,-20.8418375273512,
-1.28966629608596E-14));
#122377=CARTESIAN_POINT('Ctrl Pts',(17.0979854521548,-20.7795917637398,
1.93414622705707E-14));
#122378=CARTESIAN_POINT('Ctrl Pts',(17.0411057216723,-20.7145765131159,
1.92346139016308E-14));
#122379=CARTESIAN_POINT('Ctrl Pts',(16.9845623465869,-20.6499457268742,
1.91283973750937E-14));
#122380=CARTESIAN_POINT('Ctrl Pts',(16.9313717910731,-20.5825772843607,
1.81649823445482E-14));
#122381=CARTESIAN_POINT('Ctrl Pts',(16.8818041708791,-20.5127177725785,
2.22044604925031E-16));
#122382=CARTESIAN_POINT('Ctrl Pts',(16.8334274591801,-20.4445367009903,
-1.72897972519719E-14));
#122383=CARTESIAN_POINT('Ctrl Pts',(16.7885013791326,-20.3739820606867,
-1.50387299598194E-15));
#122384=CARTESIAN_POINT('Ctrl Pts',(16.747324449976,-20.3012692713431,-7.63278329429795E-16));
#122385=CARTESIAN_POINT('Ctrl Pts',(16.7339895188709,-20.2777216184167,
-5.23440656792113E-16));
#122386=CARTESIAN_POINT('Ctrl Pts',(16.7210481787122,-20.2539475653132,
1.14141009925036E-15));
#122387=CARTESIAN_POINT('Ctrl Pts',(16.708511751901,-20.2299543047592,-1.69309011255336E-15));
#122388=CARTESIAN_POINT('Ctrl Pts',(16.6986550608892,-20.2110897463642,
-3.79685699442959E-15));
#122389=CARTESIAN_POINT('Ctrl Pts',(16.689048690518,-20.1920896772321,1.29326085042157E-14));
#122390=CARTESIAN_POINT('Ctrl Pts',(16.6796984128078,-20.1729575913137,
-3.7470027081099E-15));
#122391=CARTESIAN_POINT('Ctrl Pts',(16.673772461475,-20.1608321963725,-1.42576522322744E-14));
#122392=CARTESIAN_POINT('Ctrl Pts',(16.6679532034413,-20.1486615485784,
2.13653143515295E-14));
#122393=CARTESIAN_POINT('Ctrl Pts',(16.6622433073212,-20.1364502099952,
2.1538326677728E-14));
#122394=CARTESIAN_POINT('Ctrl Pts',(16.6271177740505,-20.0613297926252,
2.2817734385698E-14));
#122395=CARTESIAN_POINT('Ctrl Pts',(16.596105677901,-19.9846276360536,-1.38567986312105E-14));
#122396=CARTESIAN_POINT('Ctrl Pts',(16.5694538163414,-19.9065723114556,
-7.46624984060418E-15));
#122397=CARTESIAN_POINT('Ctrl Pts',(16.5428019547817,-19.8285169868576,
-3.91519935858294E-16));
#122398=CARTESIAN_POINT('Ctrl Pts',(16.5205098557042,-19.7491077644459,
1.50329598798952E-14));
#122399=CARTESIAN_POINT('Ctrl Pts',(16.502878625203,-19.66856395302,1.87905246917808E-14));
#122400=CARTESIAN_POINT('Ctrl Pts',(16.4850541528343,-19.5871373650609,
2.27955343740806E-14));
#122401=CARTESIAN_POINT('Ctrl Pts',(16.4719940148662,-19.5045499555443,
7.18569780110884E-15));
#122402=CARTESIAN_POINT('Ctrl Pts',(16.4636225525689,-19.4211931726568,
1.68198788230711E-14));
#122403=CARTESIAN_POINT('Ctrl Pts',(16.4601640820937,-19.3867563010228,
2.08538337015049E-14));
#122404=CARTESIAN_POINT('Ctrl Pts',(16.4575064389052,-19.3521882740751,
-1.67355792731723E-14));
#122405=CARTESIAN_POINT('Ctrl Pts',(16.4556467099008,-19.3175176204782,
-1.34892097491957E-14));
#122406=CARTESIAN_POINT('Ctrl Pts',(16.4549147504963,-19.3038718092329,
-1.22694028264887E-14));
#122407=CARTESIAN_POINT('Ctrl Pts',(16.4543064087743,-19.2902081093511,
1.29130876272536E-14));
#122408=CARTESIAN_POINT('Ctrl Pts',(16.4538219778623,-19.2765459176976,
1.27398092075737E-14));
#122409=CARTESIAN_POINT('Ctrl Pts',(16.4509249680159,-19.194842824923,1.16962727565706E-14));
#122410=CARTESIAN_POINT('Ctrl Pts',(16.4524464982906,-19.1130624309727,
8.72830971514544E-15));
#122411=CARTESIAN_POINT('Ctrl Pts',(16.458252360817,-19.0315664983848,-5.74540415243519E-15));
#122412=CARTESIAN_POINT('Ctrl Pts',(16.4640582233434,-18.9500705657969,
-2.02191180200158E-14));
#122413=CARTESIAN_POINT('Ctrl Pts',(16.474148825966,-18.868858075135,1.49310499479369E-14));
#122414=CARTESIAN_POINT('Ctrl Pts',(16.4884408456005,-18.7883024616738,
1.04360964314765E-14));
#122415=CARTESIAN_POINT('Ctrl Pts',(16.5025319927713,-18.7088790468066,
6.1238295247487E-15));
#122416=CARTESIAN_POINT('Ctrl Pts',(16.5207077570521,-18.6300932899197,
-1.34620945332921E-14));
#122417=CARTESIAN_POINT('Ctrl Pts',(16.5429310587135,-18.5523284952265,
1.63757896132211E-15));
#122418=CARTESIAN_POINT('Ctrl Pts',(16.5522282722733,-18.5197952598546,
7.80572654577075E-15));
#122419=CARTESIAN_POINT('Ctrl Pts',(16.5622343667201,-18.4874410976137,
4.24674998370723E-15));
#122420=CARTESIAN_POINT('Ctrl Pts',(16.572948601838,-18.4552959778321,1.74860126378462E-14));
#122421=CARTESIAN_POINT('Ctrl Pts',(16.578489270918,-18.4386727220153,2.43262322813947E-14));
#122422=CARTESIAN_POINT('Ctrl Pts',(16.5842201970324,-18.4221033375436,
-1.47712113728087E-14));
#122423=CARTESIAN_POINT('Ctrl Pts',(16.5901333946024,-18.4056133356731,
-1.04638520070921E-14));
#122424=CARTESIAN_POINT('Ctrl Pts',(16.6168665563098,-18.3310631652543,
9.11922743263435E-15));
#122425=CARTESIAN_POINT('Ctrl Pts',(16.6473525954954,-18.2580371498547,
2.59274245153824E-14));
#122426=CARTESIAN_POINT('Ctrl Pts',(16.6815326594994,-18.186894548015,5.71764857681956E-15));
#122427=CARTESIAN_POINT('Ctrl Pts',(16.7078448582386,-18.1321281708012,
-9.84006485838118E-15));
#122428=CARTESIAN_POINT('Ctrl Pts',(16.7363470804512,-18.0784782971011,
-1.13436528624218E-14));
#122429=CARTESIAN_POINT('Ctrl Pts',(16.7670276804213,-18.0261235050124,
-7.43849426498855E-15));
#122430=CARTESIAN_POINT('Ctrl Pts',(16.7762619506765,-18.01036571997,-6.04644969543337E-15));
#122431=CARTESIAN_POINT('Ctrl Pts',(16.7856936431618,-17.9947253587034,
4.29525693792424E-15));
#122432=CARTESIAN_POINT('Ctrl Pts',(16.795322651707,-17.9792075715296,2.3037127760972E-15));
#122433=CARTESIAN_POINT('Ctrl Pts',(16.8035475707392,-17.9659525679159,
4.3176325519934E-16));
#122434=CARTESIAN_POINT('Ctrl Pts',(16.8119141895608,-17.9527907636739,
4.11143789873392E-15));
#122435=CARTESIAN_POINT('Ctrl Pts',(16.8204178980527,-17.9397316712593,
3.41393580072236E-15));
#122436=CARTESIAN_POINT('Ctrl Pts',(16.8615694249279,-17.8765355265444,
-7.90562951105595E-16));
#122437=CARTESIAN_POINT('Ctrl Pts',(16.9059580734959,-17.8156943310143,
-1.38901968370523E-14));
#122438=CARTESIAN_POINT('Ctrl Pts',(16.9535504683774,-17.7575478141846,
-2.41473507855972E-15));
#122439=CARTESIAN_POINT('Ctrl Pts',(16.9976826813803,-17.7036288115269,
8.6369744883514E-15));
#122440=CARTESIAN_POINT('Ctrl Pts',(17.044570268779,-17.6520267822693,-9.3252529599055E-15));
#122441=CARTESIAN_POINT('Ctrl Pts',(17.0942091882108,-17.6030457893103,
-4.27435864480685E-15));
#122442=CARTESIAN_POINT('Ctrl Pts',(17.0997977486715,-17.5975313010074,
-3.76768770885319E-15));
#122443=CARTESIAN_POINT('Ctrl Pts',(17.10542120347,-17.592050073031,-7.85819778827449E-15));
#122444=CARTESIAN_POINT('Ctrl Pts',(17.1110791840834,-17.5866022544178,
-1.97064586870965E-14));
#122445=CARTESIAN_POINT('Ctrl Pts',(-17.1175855514924,-17.590827960842,
-0.00214194799035405));
#122446=CARTESIAN_POINT('Ctrl Pts',(-16.6641678381752,-18.1292310858663,
-0.0445525400540117));
#122447=CARTESIAN_POINT('Ctrl Pts',(-16.345912932243,-19.6852113602882,
-0.129355067678147));
#122448=CARTESIAN_POINT('Ctrl Pts',(-18.0613969831487,-21.3602251232166,
-0.256549530862762));
#122449=CARTESIAN_POINT('Ctrl Pts',(-20.393346844718,-20.8193459211516,
-0.383725337544195));
#122450=CARTESIAN_POINT('Ctrl Pts',(-21.203092563641,-18.5684056721843,
-0.510901144225632));
#122451=CARTESIAN_POINT('Ctrl Pts',(-19.7475288416972,-16.6677876400165,
-0.638076950907064));
#122452=CARTESIAN_POINT('Ctrl Pts',(-17.3621513300928,-16.8636225363617,
-0.765252757588499));
#122453=CARTESIAN_POINT('Ctrl Pts',(-16.2353411818156,-18.9749835879209,
-0.892428564269934));
#122454=CARTESIAN_POINT('Ctrl Pts',(-17.4009050866724,-21.0654820647258,
-1.01960437095136));
#122455=CARTESIAN_POINT('Ctrl Pts',(-19.7894958141682,-21.2168759594155,
-1.1467801776328));
#122456=CARTESIAN_POINT('Ctrl Pts',(-21.2097372485274,-19.2904469218172,
-1.27395598431423));
#122457=CARTESIAN_POINT('Ctrl Pts',(-20.3586420669921,-17.0534826027649,
-1.40113179099567));
#122458=CARTESIAN_POINT('Ctrl Pts',(-18.0170393273216,-16.558306372611,
-1.5283075976771));
#122459=CARTESIAN_POINT('Ctrl Pts',(-16.3332031410643,-18.2591870619742,
-1.65548340435853));
#122460=CARTESIAN_POINT('Ctrl Pts',(-16.8519492516291,-20.5956849881885,
-1.78265921103997));
#122461=CARTESIAN_POINT('Ctrl Pts',(-19.097360012485,-21.424201689821,-1.9098350177214));
#122462=CARTESIAN_POINT('Ctrl Pts',(-21.0094105654639,-19.9846279595186,
-2.03701082440284));
#122463=CARTESIAN_POINT('Ctrl Pts',(-20.8339131261131,-17.5976815579533,
-2.16418663108427));
#122464=CARTESIAN_POINT('Ctrl Pts',(-18.7318757425753,-16.4532385853486,
-2.29136243776571));
#122465=CARTESIAN_POINT('Ctrl Pts',(-16.6317872262606,-17.6012539556073,
-2.41853824444714));
#122466=CARTESIAN_POINT('Ctrl Pts',(-16.460348455506,-19.9884950701948,
-2.54571405112858));
#122467=CARTESIAN_POINT('Ctrl Pts',(-18.3748438561772,-21.4248162457191,
-2.67288985781001));
#122468=CARTESIAN_POINT('Ctrl Pts',(-20.6188427280565,-20.592482019073,
-2.80006566449145));
#122469=CARTESIAN_POINT('Ctrl Pts',(-21.1336153829609,-18.2551073477921,
-2.92724147117288));
#122470=CARTESIAN_POINT('Ctrl Pts',(-19.4468898611942,-16.5570884370688,
-3.05441727785431));
#122471=CARTESIAN_POINT('Ctrl Pts',(-17.1061321385776,-17.056252237145,
-3.18159308453575));
#122472=CARTESIAN_POINT('Ctrl Pts',(-16.2588421420139,-19.2946469479328,
-3.30876889121718));
#122473=CARTESIAN_POINT('Ctrl Pts',(-17.6823558544925,-21.2186843501945,
-3.43594469789862));
#122474=CARTESIAN_POINT('Ctrl Pts',(-20.0706877980967,-21.0631795478994,
-3.56312050458005));
#122475=CARTESIAN_POINT('Ctrl Pts',(-21.2326916511383,-18.970798544754,
-3.69029631126149));
#122476=CARTESIAN_POINT('Ctrl Pts',(-20.1023010005601,-16.8611710436873,
-3.81747211794292));
#122477=CARTESIAN_POINT('Ctrl Pts',(-17.7165791083032,-16.6697493384941,
-3.94464792462435));
#122478=CARTESIAN_POINT('Ctrl Pts',(-16.2642777359172,-18.5721509628136,
-4.07182373130579));
#122479=CARTESIAN_POINT('Ctrl Pts',(-17.077793252575,-20.8230405026448,
-4.19899953798722));
#122480=CARTESIAN_POINT('Ctrl Pts',(-19.4107756642115,-21.3573665111786,
-4.32617534466866));
#122481=CARTESIAN_POINT('Ctrl Pts',(-21.1228584093689,-19.6849180395844,
-4.45335115135009));
#122482=CARTESIAN_POINT('Ctrl Pts',(-20.6433118332049,-17.3400627566978,
-4.58052695803153));
#122483=CARTESIAN_POINT('Ctrl Pts',(-18.4120901553326,-16.474059846431,
-4.70770276471296));
#122484=CARTESIAN_POINT('Ctrl Pts',(-16.4762007799643,-17.8814132287533,
-4.8348785713944));
#122485=CARTESIAN_POINT('Ctrl Pts',(-16.6117020541549,-20.2709635255851,
-4.96205437807583));
#122486=CARTESIAN_POINT('Ctrl Pts',(-18.694279968992,-21.4504466518017,
-5.08923018475726));
#122487=CARTESIAN_POINT('Ctrl Pts',(-20.8132985469758,-20.3377600460781,
-5.2164059914387));
#122488=CARTESIAN_POINT('Ctrl Pts',(-21.0246897639318,-17.9537246080465,
-5.34358179812013));
#122489=CARTESIAN_POINT('Ctrl Pts',(-19.1345152987216,-16.4855448821736,
-5.47075760480157));
#122490=CARTESIAN_POINT('Ctrl Pts',(-16.8768929057173,-17.2801846414369,
-5.597933411483));
#122491=CARTESIAN_POINT('Ctrl Pts',(-16.3230510066515,-19.6086112276183,
-5.72510921816443));
#122492=CARTESIAN_POINT('Ctrl Pts',(-17.9811051686122,-21.3346377663488,
-5.85228502484587));
#122493=CARTESIAN_POINT('Ctrl Pts',(-20.3298936084476,-20.8747420376322,
-5.97946083152731));
#122494=CARTESIAN_POINT('Ctrl Pts',(-21.2145487148608,-18.6508498282177,
-6.10663663820873));
#122495=CARTESIAN_POINT('Ctrl Pts',(-19.8234543356058,-16.7032442099259,
-6.23381244489018));
#122496=CARTESIAN_POINT('Ctrl Pts',(-17.4328532225945,-16.8187324555017,
-6.36098825157161));
#122497=CARTESIAN_POINT('Ctrl Pts',(-16.2359735195759,-18.8913612676384,
-6.48816405825305));
#122498=CARTESIAN_POINT('Ctrl Pts',(-17.3308780673371,-21.0196223530527,
-6.61533986493447));
#122499=CARTESIAN_POINT('Ctrl Pts',(-19.7130599007477,-21.2509682606574,
-6.74251567161592));
#122500=CARTESIAN_POINT('Ctrl Pts',(-21.1970150425329,-19.3731534791717,
-6.86969147829734));
#122501=CARTESIAN_POINT('Ctrl Pts',(-20.4213067547485,-17.1089565202789,
-6.99686728497878));
#122502=CARTESIAN_POINT('Ctrl Pts',(-18.0975992455503,-16.5356375618508,
-7.12404309166021));
#122503=CARTESIAN_POINT('Ctrl Pts',(-16.3577499290741,-18.1791811640576,
-7.25121889834165));
#122504=CARTESIAN_POINT('Ctrl Pts',(-16.7979625659597,-20.5317380816948,
-7.37839470502308));
#122505=CARTESIAN_POINT('Ctrl Pts',(-19.014369384542,-21.4349833589804,
-7.50557051170451));
#122506=CARTESIAN_POINT('Ctrl Pts',(-20.9735546944935,-20.0602455157292,
-7.63274631838594));
#122507=CARTESIAN_POINT('Ctrl Pts',(-20.8780875746881,-17.6687611972708,
-7.75992212506739));
#122508=CARTESIAN_POINT('Ctrl Pts',(-18.8155531821895,-16.4545688335337,
-7.88709793174882));
#122509=CARTESIAN_POINT('Ctrl Pts',(-16.6781988067934,-17.5316145569697,
-8.01427373843027));
#122510=CARTESIAN_POINT('Ctrl Pts',(-16.4269144287518,-19.9117757653229,
-8.14144954511167));
#122511=CARTESIAN_POINT('Ctrl Pts',(-18.2922378684508,-21.4114022793946,
-8.26862535179315));
#122512=CARTESIAN_POINT('Ctrl Pts',(-20.5628506449959,-20.6546798498427,
-8.39580115847454));
#122513=CARTESIAN_POINT('Ctrl Pts',(-21.15560646603,-18.3358543382901,-8.52297696515602));
#122514=CARTESIAN_POINT('Ctrl Pts',(-19.5266886563297,-16.5823042290437,
-8.65015277183742));
#122515=CARTESIAN_POINT('Ctrl Pts',(-17.1705282042537,-17.0028029097426,
-8.77732857851889));
#122516=CARTESIAN_POINT('Ctrl Pts',(-16.2487560847711,-19.2115689399372,
-8.90450438520028));
#122517=CARTESIAN_POINT('Ctrl Pts',(-17.6070410058773,-21.1821965784047,
-9.03168019188174));
#122518=CARTESIAN_POINT('Ctrl Pts',(-19.9992408571273,-21.1067572777967,
-9.15885599856315));
#122519=CARTESIAN_POINT('Ctrl Pts',(-21.2306607516671,-19.0544619141298,
-9.28603180524462));
#122520=CARTESIAN_POINT('Ctrl Pts',(-20.1715493667948,-16.9081641037524,
-9.41320761192604));
#122521=CARTESIAN_POINT('Ctrl Pts',(-17.7935756622645,-16.6369588734199,
-9.54038341860746));
#122522=CARTESIAN_POINT('Ctrl Pts',(-16.2783829182894,-18.4896601890674,
-9.66755922528891));
#122523=CARTESIAN_POINT('Ctrl Pts',(-17.0160664339986,-20.7665295852005,
-9.79473503197033));
#122524=CARTESIAN_POINT('Ctrl Pts',(-19.3298473695317,-21.3786807093197,
-9.92191083865178));
#122525=CARTESIAN_POINT('Ctrl Pts',(-21.0969753259781,-19.7645028994292,
-10.0490866453332));
#122526=CARTESIAN_POINT('Ctrl Pts',(-20.6962200836287,-17.4049041089298,
-10.1762624520146));
#122527=CARTESIAN_POINT('Ctrl Pts',(-18.4952497036636,-16.4646697748868,
-10.3034382586961));
#122528=CARTESIAN_POINT('Ctrl Pts',(-16.5133179020725,-17.8064065412604,
-10.4306140653775));
#122529=CARTESIAN_POINT('Ctrl Pts',(-16.5687240942544,-20.1991542024786,
-10.5577898720589));
#122530=CARTESIAN_POINT('Ctrl Pts',(-18.6106365377785,-21.4477152900423,
-10.6849656787404));
#122531=CARTESIAN_POINT('Ctrl Pts',(-20.7657273010908,-20.4066125005527,
-10.8121414854218));
#122532=CARTESIAN_POINT('Ctrl Pts',(-21.0568343688704,-18.0309930252399,
-10.9393172921033));
#122533=CARTESIAN_POINT('Ctrl Pts',(-19.2168850745718,-16.5003402851297,
-11.0664930987847));
#122534=CARTESIAN_POINT('Ctrl Pts',(-16.9339186955814,-17.2189331662498,
-11.1936689054661));
#122535=CARTESIAN_POINT('Ctrl Pts',(-16.302415187749,-19.5275073010768,
-11.3208447121476));
#122536=CARTESIAN_POINT('Ctrl Pts',(-17.9017398239826,-21.3080892071774,
-11.448020518829));
#122537=CARTESIAN_POINT('Ctrl Pts',(-20.26461151582,-20.9271055010812,-11.5751963255104));
#122538=CARTESIAN_POINT('Ctrl Pts',(-21.2232421423571,-18.7340850866159,
-11.7023721321919));
#122539=CARTESIAN_POINT('Ctrl Pts',(-19.8981476030732,-16.7409880798555,
-11.8295479388733));
#122540=CARTESIAN_POINT('Ctrl Pts',(-17.5050198931187,-16.7763572789512,
-11.9567237455547));
#122541=CARTESIAN_POINT('Ctrl Pts',(-16.2394051521196,-18.8077436389928,
-12.0838995522362));
#122542=CARTESIAN_POINT('Ctrl Pts',(-17.2624263520327,-20.9714762566988,
-12.2110753589176));
#122543=CARTESIAN_POINT('Ctrl Pts',(-19.6355250377943,-21.2824647517163,
-12.3382511655991));
#122544=CARTESIAN_POINT('Ctrl Pts',(-21.181530456334,-19.4553964819894,
-12.4654269722804));
#122545=CARTESIAN_POINT('Ctrl Pts',(-20.4820785920598,-17.1664931843466,
-12.5926027789619));
#122546=CARTESIAN_POINT('Ctrl Pts',(-18.1788731175643,-16.5156815690145,
-12.7197785856433));
#122547=CARTESIAN_POINT('Ctrl Pts',(-16.3849621026435,-18.1000408991359,
-12.8469543923248));
#122548=CARTESIAN_POINT('Ctrl Pts',(-16.7461475608124,-20.4660198257546,
-12.9741301990062));
#122549=CARTESIAN_POINT('Ctrl Pts',(-18.9310642518988,-21.4429795329118,
-13.1013060056876));
#122550=CARTESIAN_POINT('Ctrl Pts',(-20.9351867230549,-20.1346201262487,
-13.2284818123691));
#122551=CARTESIAN_POINT('Ctrl Pts',(-20.9198569968642,-17.7412801554356,
-13.3556576190505));
#122552=CARTESIAN_POINT('Ctrl Pts',(-18.8991391456364,-16.4587004962619,
-13.4828334257319));
#122553=CARTESIAN_POINT('Ctrl Pts',(-16.7269163779785,-17.463568380148,
-13.6100092324134));
#122554=CARTESIAN_POINT('Ctrl Pts',(-16.3960682598664,-19.8339798927631,
-13.7371850390948));
#122555=CARTESIAN_POINT('Ctrl Pts',(-18.210127404918,-21.395229595614,-13.8643608457763));
#122556=CARTESIAN_POINT('Ctrl Pts',(-20.5048071407569,-20.71496778842,-13.9915366524577));
#122557=CARTESIAN_POINT('Ctrl Pts',(-21.174881233638,-18.417292457472,-14.1187124591391));
#122558=CARTESIAN_POINT('Ctrl Pts',(-19.6055982928313,-16.6101781091006,
-14.2458882658205));
#122559=CARTESIAN_POINT('Ctrl Pts',(-17.236678015843,-16.9515399957704,
-14.373064072502));
#122560=CARTESIAN_POINT('Ctrl Pts',(-16.2414577250354,-19.12819977377,-14.5002398791834));
#122561=CARTESIAN_POINT('Ctrl Pts',(-17.5329902668867,-21.1432071955271,
-14.6274156858649));
#122562=CARTESIAN_POINT('Ctrl Pts',(-19.9263746957985,-21.1479180170447,
-14.7545914925463));
#122563=CARTESIAN_POINT('Ctrl Pts',(-21.2258293484353,-19.1380103519671,
-14.8817672992277));
#122564=CARTESIAN_POINT('Ctrl Pts',(-20.2391852342543,-16.9574497340641,
-15.0089431059091));
#122565=CARTESIAN_POINT('Ctrl Pts',(-17.8716270899769,-16.6067651894063,
-15.1361189125906));
#122566=CARTESIAN_POINT('Ctrl Pts',(-16.2952425657462,-18.4076880217795,
-15.263294719272));
#122567=CARTESIAN_POINT('Ctrl Pts',(-16.9562666210861,-20.7079833103585,
-15.3904705259535));
#122568=CARTESIAN_POINT('Ctrl Pts',(-19.2482507130021,-21.3972729002994,
-15.5176463326349));
#122569=CARTESIAN_POINT('Ctrl Pts',(-21.0684416937376,-19.8431763749684,
-15.6448221393163));
#122570=CARTESIAN_POINT('Ctrl Pts',(-20.746927312261,-17.4714808382477,
-15.7719979459977));
#122571=CARTESIAN_POINT('Ctrl Pts',(-18.5786770581442,-16.4580697410522,
-15.8991737526792));
#122572=CARTESIAN_POINT('Ctrl Pts',(-16.552925962751,-17.7326848656722,
-16.0263495593606));
#122573=CARTESIAN_POINT('Ctrl Pts',(-16.5281749238118,-20.1259459468057,
-16.1535253660421));
#122574=CARTESIAN_POINT('Ctrl Pts',(-18.5271314833305,-21.4421844850479,
-16.2807011727235));
#122575=CARTESIAN_POINT('Ctrl Pts',(-20.7158770671853,-20.4738333165386,
-16.4078769794049));
#122576=CARTESIAN_POINT('Ctrl Pts',(-21.0863734510612,-18.1092945357334,
-16.5350527860864));
#122577=CARTESIAN_POINT('Ctrl Pts',(-19.298713198351,-16.5178857141929,
-16.6622285927678));
#122578=CARTESIAN_POINT('Ctrl Pts',(-16.9929636362077,-17.1596256717093,
-16.7894043994492));
#122579=CARTESIAN_POINT('Ctrl Pts',(-16.2845068769401,-19.4457578281354,
-16.9165802061307));
#122580=CARTESIAN_POINT('Ctrl Pts',(-17.8233080253906,-21.2788978233141,
-17.0437560128121));
#122581=CARTESIAN_POINT('Ctrl Pts',(-20.1976125366265,-20.9772534891692,
-17.1709318194935));
#122582=CARTESIAN_POINT('Ctrl Pts',(-21.2291433875466,-18.8175647801194,
-17.298107626175));
#122583=CARTESIAN_POINT('Ctrl Pts',(-19.9715350464571,-16.7812120413194,
-17.4252834328564));
#122584=CARTESIAN_POINT('Ctrl Pts',(-17.5785651103304,-16.7364225203127,
-17.5524592395378));
#122585=CARTESIAN_POINT('Ctrl Pts',(-16.2456349710989,-18.7242878226724,
-17.6796350462193));
#122586=CARTESIAN_POINT('Ctrl Pts',(-17.1956253005315,-20.9210649143176,
-17.8068108529007));
#122587=CARTESIAN_POINT('Ctrl Pts',(-19.5569789344254,-21.31134716103,-17.9339866595822));
#122588=CARTESIAN_POINT('Ctrl Pts',(-21.163300475815,-19.5370748250935,
-18.0611624662636));
#122589=CARTESIAN_POINT('Ctrl Pts',(-20.5408896100412,-17.2260326509801,
-18.188338272945));
#122590=CARTESIAN_POINT('Ctrl Pts',(-18.2607696752627,-16.4984583939631,
-18.3155140796264));
#122591=CARTESIAN_POINT('Ctrl Pts',(-16.4148091914615,-18.0218562765459,
-18.4426898863079));
#122592=CARTESIAN_POINT('Ctrl Pts',(-16.6965623292452,-20.3986032941145,
-18.5698656929893));
#122593=CARTESIAN_POINT('Ctrl Pts',(-18.8475380723677,-21.4481815757617,
-18.6970414996708));
#122594=CARTESIAN_POINT('Ctrl Pts',(-20.894349680935,-20.2076681919521,
-18.8242173063522));
#122595=CARTESIAN_POINT('Ctrl Pts',(-20.9591745439093,-17.8151571779635,
-18.9513931130336));
#122596=CARTESIAN_POINT('Ctrl Pts',(-18.9825398722896,-16.4656288920389,
-19.078568919715));
#122597=CARTESIAN_POINT('Ctrl Pts',(-16.7778852948647,-17.3971917774822,
-19.2057447263965));
#122598=CARTESIAN_POINT('Ctrl Pts',(-16.3678445475033,-19.7551947020895,
-19.3329205330779));
#122599=CARTESIAN_POINT('Ctrl Pts',(-18.1286045709649,-21.3763163446451,
-19.4600963397593));
#122600=CARTESIAN_POINT('Ctrl Pts',(-20.4447773190769,-20.773278200954,
-19.5872721464408));
#122601=CARTESIAN_POINT('Ctrl Pts',(-21.1914180721045,-18.4993303685776,
-19.7144479531222));
#122602=CARTESIAN_POINT('Ctrl Pts',(-19.6835302447416,-16.6406787897749,
-19.8416237598037));
#122603=CARTESIAN_POINT('Ctrl Pts',(-17.304507398182,-16.9025210366613,
-19.9687995664851));
#122604=CARTESIAN_POINT('Ctrl Pts',(-16.2369552011117,-19.0446328885181,
-20.0959753731665));
#122605=CARTESIAN_POINT('Ctrl Pts',(-17.4602867931939,-21.1017600821981,
-20.223151179848));
#122606=CARTESIAN_POINT('Ctrl Pts',(-19.8521708689288,-21.1866153140319,
-20.3503269865294));
#122607=CARTESIAN_POINT('Ctrl Pts',(-21.2182032059767,-19.221350684525,
-20.4775027932109));
#122608=CARTESIAN_POINT('Ctrl Pts',(-20.3051320707828,-17.0089716056813,
-20.6046785998922));
#122609=CARTESIAN_POINT('Ctrl Pts',(-17.9506471225061,-16.5792041686457,
-20.7318544065737));
#122610=CARTESIAN_POINT('Ctrl Pts',(-16.3148352980017,-18.3263225287329,
-20.8590302132551));
#122611=CARTESIAN_POINT('Ctrl Pts',(-16.8984656481068,-20.647474826016,
-20.9862060199366));
#122612=CARTESIAN_POINT('Ctrl Pts',(-19.1660680562885,-21.4131078237249,
-21.113381826618));
#122613=CARTESIAN_POINT('Ctrl Pts',(-21.0373071781416,-19.9208779742462,
-21.2405576332995));
#122614=CARTESIAN_POINT('Ctrl Pts',(-20.7953426154092,-17.5396647859301,
-21.3677334399809));
#122615=CARTESIAN_POINT('Ctrl Pts',(-18.6623441981192,-16.4543701936005,
-21.4949092466623));
#122616=CARTESIAN_POINT('Ctrl Pts',(-16.5948542065943,-17.6601323237235,
-21.6220850533437));
#122617=CARTESIAN_POINT('Ctrl Pts',(-16.4903435139124,-20.0518037409453,
-21.7492608600252));
#122618=CARTESIAN_POINT('Ctrl Pts',(-18.4433885276789,-21.4331202535291,
-21.8764366667066));
#122619=CARTESIAN_POINT('Ctrl Pts',(-20.6647168408145,-20.5407968853708,
-22.0036124733881));
#122620=CARTESIAN_POINT('Ctrl Pts',(-21.1114425640841,-18.1855248151863,
-22.1307882800695));
#122621=CARTESIAN_POINT('Ctrl Pts',(-19.9599076846608,-17.0924953497883,
-22.2155721511904));
#122622=CARTESIAN_POINT('Ctrl Pts',(-19.2802416510892,-16.9106266592565,
-22.2579640867509));
#122623=CARTESIAN_POINT('Ctrl Pts',(-17.0028272034401,-17.4941907062238,
0.0844764445356071));
#122624=CARTESIAN_POINT('Ctrl Pts',(-16.5172188178569,-18.0708180956198,
0.0420658524719494));
#122625=CARTESIAN_POINT('Ctrl Pts',(-16.1763692071458,-19.7372661563571,
-0.0427366751521866));
#122626=CARTESIAN_POINT('Ctrl Pts',(-18.0136451140781,-21.531198562073,
-0.1699311383368));
#122627=CARTESIAN_POINT('Ctrl Pts',(-20.5111532049132,-20.9519193050085,
-0.297106945018234));
#122628=CARTESIAN_POINT('Ctrl Pts',(-21.3783873242474,-18.5411721545534,
-0.424282751699668));
#122629=CARTESIAN_POINT('Ctrl Pts',(-19.8194849515203,-16.5056185643353,
-0.551458558381103));
#122630=CARTESIAN_POINT('Ctrl Pts',(-17.2647560814413,-16.7153568808188,
-0.678634365062537));
#122631=CARTESIAN_POINT('Ctrl Pts',(-16.0579473465983,-18.9766153220251,
-0.805810171743972));
#122632=CARTESIAN_POINT('Ctrl Pts',(-17.306261185047,-21.2155300370204,
-0.932985978425408));
#122633=CARTESIAN_POINT('Ctrl Pts',(-19.8644313952761,-21.3776722353249,
-1.06016178510684));
#122634=CARTESIAN_POINT('Ctrl Pts',(-21.3855037526656,-19.3144751713091,
-1.18733759178828));
#122635=CARTESIAN_POINT('Ctrl Pts',(-20.4739845399306,-16.9186961805966,
-1.31451339846971));
#122636=CARTESIAN_POINT('Ctrl Pts',(-17.9661382589161,-16.3883646063293,
-1.44168920515115));
#122637=CARTESIAN_POINT('Ctrl Pts',(-16.1627570764457,-18.2100003769934,
-1.56886501183258));
#122638=CARTESIAN_POINT('Ctrl Pts',(-16.7183318894278,-20.7123794251487,
-1.69604081851402));
#122639=CARTESIAN_POINT('Ctrl Pts',(-19.1231569823275,-21.5997171847722,
-1.82321662519545));
#122640=CARTESIAN_POINT('Ctrl Pts',(-21.1709547522747,-20.0579400230779,
-1.95039243187689));
#122641=CARTESIAN_POINT('Ctrl Pts',(-20.9829977631806,-17.5015308787203,
-2.07756823855832));
#122642=CARTESIAN_POINT('Ctrl Pts',(-18.7317249295996,-16.2758374662316,
-2.20474404523976));
#122643=CARTESIAN_POINT('Ctrl Pts',(-16.4825393242813,-17.5053569009653,
-2.33191985192118));
#122644=CARTESIAN_POINT('Ctrl Pts',(-16.2989291514817,-20.062081681679,
-2.45909565860262));
#122645=CARTESIAN_POINT('Ctrl Pts',(-18.3493453426023,-21.6003753714481,
-2.58627146528406));
#122646=CARTESIAN_POINT('Ctrl Pts',(-20.7526583085904,-20.708949059251,
-2.71344727196549));
#122647=CARTESIAN_POINT('Ctrl Pts',(-21.3039775679586,-18.2056310209682,
-2.84062307864693));
#122648=CARTESIAN_POINT('Ctrl Pts',(-19.4975019198092,-16.3870602026966,
-2.96779888532836));
#122649=CARTESIAN_POINT('Ctrl Pts',(-16.9905606483594,-16.9216624468904,
-3.09497469200979));
#122650=CARTESIAN_POINT('Ctrl Pts',(-16.0831167720671,-19.3189733808883,
-3.22215049869123));
#122651=CARTESIAN_POINT('Ctrl Pts',(-17.6076937249943,-21.3796090139306,
-3.34932630537266));
#122652=CARTESIAN_POINT('Ctrl Pts',(-20.1655867788085,-21.2130640515812,
-3.4765021120541));
#122653=CARTESIAN_POINT('Ctrl Pts',(-21.4100878173515,-18.9721331591184,
-3.60367791873553));
#122654=CARTESIAN_POINT('Ctrl Pts',(-20.1994443802222,-16.7127313428988,
-3.73085372541697));
#122655=CARTESIAN_POINT('Ctrl Pts',(-17.6443466799723,-16.507719534815,
-3.8580295320984));
#122656=CARTESIAN_POINT('Ctrl Pts',(-16.0889382693367,-18.545183344418,
-3.98520533877984));
#122657=CARTESIAN_POINT('Ctrl Pts',(-16.9602098255379,-20.95587618561,-4.11238114546127));
#122658=CARTESIAN_POINT('Ctrl Pts',(-19.458823772974,-21.5281370010973,
-4.2395569521427));
#122659=CARTESIAN_POINT('Ctrl Pts',(-21.2924568963431,-19.7369520111678,
-4.36673275882414));
#122660=CARTESIAN_POINT('Ctrl Pts',(-20.7788646130614,-17.2256222706107,
-4.49390856550557));
#122661=CARTESIAN_POINT('Ctrl Pts',(-18.3892359659074,-16.2981369456807,
-4.62108437218701));
#122662=CARTESIAN_POINT('Ctrl Pts',(-16.3159069215641,-17.8054062557716,
-4.74826017886844));
#122663=CARTESIAN_POINT('Ctrl Pts',(-16.4610281929029,-20.3646041605579,
-4.87543598554988));
#122664=CARTESIAN_POINT('Ctrl Pts',(-18.6914600207125,-21.6278254241348,
-5.00261179223131));
#122665=CARTESIAN_POINT('Ctrl Pts',(-20.9609196391894,-20.436142941524,
-5.12978759891275));
#122666=CARTESIAN_POINT('Ctrl Pts',(-21.187318706931,-17.8828514263649,
-5.25696340559418));
#122667=CARTESIAN_POINT('Ctrl Pts',(-19.1629501311951,-16.3104373686715,
-5.38413921227561));
#122668=CARTESIAN_POINT('Ctrl Pts',(-16.7450464337354,-17.1614930713546,
-5.51131501895704));
#122669=CARTESIAN_POINT('Ctrl Pts',(-16.1518841849428,-19.6552277496765,
-5.63849082563848));
#122670=CARTESIAN_POINT('Ctrl Pts',(-17.9276529322832,-21.503794614907,
-5.76566663231992));
#122671=CARTESIAN_POINT('Ctrl Pts',(-20.4431950667104,-21.0112483031962,
-5.89284243900135));
#122672=CARTESIAN_POINT('Ctrl Pts',(-21.3906568120407,-18.629469484667,
-6.02001824568278));
#122673=CARTESIAN_POINT('Ctrl Pts',(-19.9008008230416,-16.5435923954545,
-6.14719405236422));
#122674=CARTESIAN_POINT('Ctrl Pts',(-17.3404774987283,-16.667279800778,
-6.27436985904566));
#122675=CARTESIAN_POINT('Ctrl Pts',(-16.0586245775708,-18.8870561831594,
-6.40154566572708));
#122676=CARTESIAN_POINT('Ctrl Pts',(-17.2312625539661,-21.1664144866242,
-6.52872147240852));
#122677=CARTESIAN_POINT('Ctrl Pts',(-19.7825688666926,-21.414184940675,
-6.65589727908996));
#122678=CARTESIAN_POINT('Ctrl Pts',(-21.3718783257522,-19.4030535320888,
-6.78307308577139));
#122679=CARTESIAN_POINT('Ctrl Pts',(-20.5410981461279,-16.9781085033506,
-6.91024889245283));
#122680=CARTESIAN_POINT('Ctrl Pts',(-18.0524175785914,-16.3640864092651,
-7.03742469913425));
#122681=CARTESIAN_POINT('Ctrl Pts',(-16.1890465789213,-18.1243144106463,
-7.1646005058157));
#122682=CARTESIAN_POINT('Ctrl Pts',(-16.6605123854672,-20.6438925682982,
-7.29177631249713));
#122683=CARTESIAN_POINT('Ctrl Pts',(-19.0342743831914,-21.6112643052322,
-7.41895211917856));
#122684=CARTESIAN_POINT('Ctrl Pts',(-21.1325532714676,-20.1389260946729,
-7.54612792586));
#122685=CARTESIAN_POINT('Ctrl Pts',(-21.0303084041777,-17.5776568611929,
-7.67330373254143));
#122686=CARTESIAN_POINT('Ctrl Pts',(-18.8213431010281,-16.277262156213,
-7.80047953922286));
#122687=CARTESIAN_POINT('Ctrl Pts',(-16.5322459238095,-17.4307734099542,
-7.92765534590431));
#122688=CARTESIAN_POINT('Ctrl Pts',(-16.2631214552256,-19.979915642092,
-8.05483115258573));
#122689=CARTESIAN_POINT('Ctrl Pts',(-18.260874691454,-21.5860090722502,
-8.18200695926717));
#122690=CARTESIAN_POINT('Ctrl Pts',(-20.6926910328048,-20.7755626636597,
-8.30918276594861));
#122691=CARTESIAN_POINT('Ctrl Pts',(-21.3275299216332,-18.2921106942249,
-8.43635857263003));
#122692=CARTESIAN_POINT('Ctrl Pts',(-19.5829660799844,-16.4140662054893,
-8.56353437931147));
#122693=CARTESIAN_POINT('Ctrl Pts',(-17.0595285527274,-16.8644184512809,
-8.69071018599291));
#122694=CARTESIAN_POINT('Ctrl Pts',(-16.0723146489239,-19.2299971980986,
-8.81788599267433));
#122695=CARTESIAN_POINT('Ctrl Pts',(-17.5270318519084,-21.3405307701129,
-8.94506179935578));
#122696=CARTESIAN_POINT('Ctrl Pts',(-20.089067417875,-21.2597356094876,
-9.07223760603719));
#122697=CARTESIAN_POINT('Ctrl Pts',(-21.4079127329105,-19.0617362613832,
-9.19941341271864));
#122698=CARTESIAN_POINT('Ctrl Pts',(-20.2736090772418,-16.7630607044602,
-9.32658921940007));
#122699=CARTESIAN_POINT('Ctrl Pts',(-17.7268096521201,-16.4726010903001,
-9.45376502608151));
#122700=CARTESIAN_POINT('Ctrl Pts',(-16.1040448578949,-18.4568360869378,
-9.58094083276294));
#122701=CARTESIAN_POINT('Ctrl Pts',(-16.8941006731258,-20.8953532404716,
-9.70811663944438));
#122702=CARTESIAN_POINT('Ctrl Pts',(-19.3721499237325,-21.5509644139779,
-9.83529244612582));
#122703=CARTESIAN_POINT('Ctrl Pts',(-21.2647362273657,-19.8221870475835,
-9.96246825280725));
#122704=CARTESIAN_POINT('Ctrl Pts',(-20.835529117596,-17.2950670749305,
-10.0896440594887));
#122705=CARTESIAN_POINT('Ctrl Pts',(-18.4782994780394,-16.2880802201732,
-10.2168198661701));
#122706=CARTESIAN_POINT('Ctrl Pts',(-16.3556591968173,-17.7250744218984,
-10.3439956728516));
#122707=CARTESIAN_POINT('Ctrl Pts',(-16.414998986037,-20.2876966899422,
-10.471171479533));
#122708=CARTESIAN_POINT('Ctrl Pts',(-18.6018782721322,-21.6249001476502,
-10.5983472862144));
#122709=CARTESIAN_POINT('Ctrl Pts',(-20.9099710431467,-20.5098836187822,
-10.7255230928959));
#122710=CARTESIAN_POINT('Ctrl Pts',(-21.2217454380686,-17.965605562844,
-10.8526988995773));
#122711=CARTESIAN_POINT('Ctrl Pts',(-19.2511678004582,-16.3262831804529,
-10.9798747062588));
#122712=CARTESIAN_POINT('Ctrl Pts',(-16.8061208049812,-17.0958930096308,
-11.1070505129402));
#122713=CARTESIAN_POINT('Ctrl Pts',(-16.1297833132563,-19.5683657994802,
-11.2342263196216));
#122714=CARTESIAN_POINT('Ctrl Pts',(-17.8426529957019,-21.4753612242825,
-11.361402126303));
#122715=CARTESIAN_POINT('Ctrl Pts',(-20.3732782313567,-21.0673293432663,
-11.4885779329845));
#122716=CARTESIAN_POINT('Ctrl Pts',(-21.3999674348234,-18.7186140819493,
-11.6157537396659));
#122717=CARTESIAN_POINT('Ctrl Pts',(-19.98079698544,-16.5840159148801,-11.7429295463474));
#122718=CARTESIAN_POINT('Ctrl Pts',(-17.4177676868637,-16.6218961722405,
-11.8701053530288));
#122719=CARTESIAN_POINT('Ctrl Pts',(-16.0622998409991,-18.7975020690164,
-11.9972811597103));
#122720=CARTESIAN_POINT('Ctrl Pts',(-17.1579510666044,-21.1148502282466,
-12.1244569663916));
#122721=CARTESIAN_POINT('Ctrl Pts',(-19.6995293679712,-21.4479175446854,
-12.2516327730731));
#122722=CARTESIAN_POINT('Ctrl Pts',(-21.3552944017355,-19.4911354279892,
-12.3788085797545));
#122723=CARTESIAN_POINT('Ctrl Pts',(-20.6061845177868,-17.0397300186315,
-12.505984386436));
#122724=CARTESIAN_POINT('Ctrl Pts',(-18.1394615396447,-16.3427136283187,
-12.6331601931174));
#122725=CARTESIAN_POINT('Ctrl Pts',(-16.2181906976602,-18.0395555334466,
-12.7603359997988));
#122726=CARTESIAN_POINT('Ctrl Pts',(-16.6050187418368,-20.5735086039467,
-12.8875118064803));
#122727=CARTESIAN_POINT('Ctrl Pts',(-18.9450549508987,-21.6198281725,-13.0146876131617));
#122728=CARTESIAN_POINT('Ctrl Pts',(-21.0914613420586,-20.2185809768753,
-13.1418634198431));
#122729=CARTESIAN_POINT('Ctrl Pts',(-21.0750432724325,-17.6553243478488,
-13.2690392265246));
#122730=CARTESIAN_POINT('Ctrl Pts',(-18.9108633018819,-16.2816871489036,
-13.396215033206));
#122731=CARTESIAN_POINT('Ctrl Pts',(-16.5844222292293,-17.3578962525319,
-13.5233908398874));
#122732=CARTESIAN_POINT('Ctrl Pts',(-16.2300853434153,-19.8965966032252,
-13.6505666465689));
#122733=CARTESIAN_POINT('Ctrl Pts',(-18.1729347445473,-21.5686881987366,
-13.7777424532503));
#122734=CARTESIAN_POINT('Ctrl Pts',(-20.6305266939199,-20.8401307818932,
-13.9049182599318));
#122735=CARTESIAN_POINT('Ctrl Pts',(-21.348173113343,-18.3793305632757,
-14.0320940666132));
#122736=CARTESIAN_POINT('Ctrl Pts',(-19.6674779551561,-16.443919008979,
-14.1592698732946));
#122737=CARTESIAN_POINT('Ctrl Pts',(-17.1303747112896,-16.8095160948814,
-14.2864456799761));
#122738=CARTESIAN_POINT('Ctrl Pts',(-16.0644981376042,-19.140709186182,
-14.4136214866575));
#122739=CARTESIAN_POINT('Ctrl Pts',(-17.4477238346954,-21.2987733117736,
-14.5407972933389));
#122740=CARTESIAN_POINT('Ctrl Pts',(-20.0110280781508,-21.3038185809918,
-14.6679731000203));
#122741=CARTESIAN_POINT('Ctrl Pts',(-21.4027383212044,-19.1512162724734,
-14.7951489067018));
#122742=CARTESIAN_POINT('Ctrl Pts',(-20.3460467951339,-16.8158453987172,
-14.9223247133832));
#122743=CARTESIAN_POINT('Ctrl Pts',(-17.8104023894363,-16.4402637869306,
-15.0495005200647));
#122744=CARTESIAN_POINT('Ctrl Pts',(-16.1221014664979,-18.3690442547039,
-15.1766763267461));
#122745=CARTESIAN_POINT('Ctrl Pts',(-16.8300553353419,-20.8326504364724,
-15.3038521334275));
#122746=CARTESIAN_POINT('Ctrl Pts',(-19.2847602618764,-21.5708765691077,
-15.4310279401089));
#122747=CARTESIAN_POINT('Ctrl Pts',(-21.2341768321763,-19.9064459953984,
-15.5582037467904));
#122748=CARTESIAN_POINT('Ctrl Pts',(-20.8898363374295,-17.3663704605105,
-15.6853795534718));
#122749=CARTESIAN_POINT('Ctrl Pts',(-18.5676498093848,-16.2810116128359,
-15.8125553601533));
#122750=CARTESIAN_POINT('Ctrl Pts',(-16.3980792563722,-17.6461188301484,
-15.9397311668347));
#122751=CARTESIAN_POINT('Ctrl Pts',(-16.3715710020456,-20.2092909686735,
-16.0669069735161));
#122752=CARTESIAN_POINT('Ctrl Pts',(-18.5124447244619,-21.618976679719,
-16.1940827801976));
#122753=CARTESIAN_POINT('Ctrl Pts',(-20.8565816609132,-20.5818768183634,
-16.321258586879));
#122754=CARTESIAN_POINT('Ctrl Pts',(-21.2533816657522,-18.0494661377238,
-16.4484343935604));
#122755=CARTESIAN_POINT('Ctrl Pts',(-19.338805362725,-16.3450742581534,
-16.5756102002418));
#122756=CARTESIAN_POINT('Ctrl Pts',(-16.869357677852,-17.0323749426676,
-16.7027860069233));
#122757=CARTESIAN_POINT('Ctrl Pts',(-16.1106035907951,-19.4808124719162,
-16.8299618136047));
#122758=CARTESIAN_POINT('Ctrl Pts',(-17.7586528828391,-21.4440973799852,
-16.9571376202862));
#122759=CARTESIAN_POINT('Ctrl Pts',(-20.3015226180088,-21.1210376189256,
-17.0843134269676));
#122760=CARTESIAN_POINT('Ctrl Pts',(-21.4062876425816,-18.8080204681591,
-17.211489233649));
#122761=CARTESIAN_POINT('Ctrl Pts',(-20.0593946159625,-16.6270956014793,
-17.3386650403305));
#122762=CARTESIAN_POINT('Ctrl Pts',(-17.4965342924651,-16.5791262206009,
-17.4658408470119));
#122763=CARTESIAN_POINT('Ctrl Pts',(-16.0689719498474,-18.7081212551652,
-17.5930166536933));
#122764=CARTESIAN_POINT('Ctrl Pts',(-17.0864074329483,-21.0608599012923,
-17.7201924603748));
#122765=CARTESIAN_POINT('Ctrl Pts',(-19.6154068351929,-21.4788504785931,
-17.8473682670562));
#122766=CARTESIAN_POINT('Ctrl Pts',(-21.3357701724232,-19.5786125758088,
-17.9745440737377));
#122767=CARTESIAN_POINT('Ctrl Pts',(-20.6691708605291,-17.1034965266906,
-18.1017198804191));
#122768=CARTESIAN_POINT('Ctrl Pts',(-18.2271723943392,-16.3242676832537,
-18.2288956871005));
#122769=CARTESIAN_POINT('Ctrl Pts',(-16.2501567990929,-17.9558201449997,
-18.3560714937819));
#122770=CARTESIAN_POINT('Ctrl Pts',(-16.5519131759471,-20.5013057937568,
-18.4832473004634));
#122771=CARTESIAN_POINT('Ctrl Pts',(-18.8555987783568,-21.6253995376139,
-18.6104231071448));
#122772=CARTESIAN_POINT('Ctrl Pts',(-21.0477250487613,-20.2968151353882,
-18.7375989138263));
#122773=CARTESIAN_POINT('Ctrl Pts',(-21.1171521931581,-17.7344463154909,
-18.8647747205077));
#122774=CARTESIAN_POINT('Ctrl Pts',(-19.000185114941,-16.2891074304433,
-18.9919505271891));
#122775=CARTESIAN_POINT('Ctrl Pts',(-16.6390097160369,-17.2868072017201,
-19.1191263338706));
#122776=CARTESIAN_POINT('Ctrl Pts',(-16.1998578710576,-19.8122180089903,
-19.246302140552));
#122777=CARTESIAN_POINT('Ctrl Pts',(-18.0856241463476,-21.5484321897643,
-19.3734779472334));
#122778=CARTESIAN_POINT('Ctrl Pts',(-20.566235017753,-20.9025809783934,
-19.5006537539149));
#122779=CARTESIAN_POINT('Ctrl Pts',(-21.3658839949308,-18.4671928068505,
-19.6278295605963));
#122780=CARTESIAN_POINT('Ctrl Pts',(-19.7509427344116,-16.4765851044279,
-19.7550053672777));
#122781=CARTESIAN_POINT('Ctrl Pts',(-17.2030196827703,-16.757017004315,
-19.8821811739592));
#122782=CARTESIAN_POINT('Ctrl Pts',(-16.0596759541972,-19.0512094179914,
-20.0093569806406));
#122783=CARTESIAN_POINT('Ctrl Pts',(-17.3698587327169,-21.2543836348827,
-20.136532787322));
#122784=CARTESIAN_POINT('Ctrl Pts',(-19.9315561044895,-21.3452632166212,
-20.2637085940035));
#122785=CARTESIAN_POINT('Ctrl Pts',(-21.394570756024,-19.2404734037209,
-20.3908844006849));
#122786=CARTESIAN_POINT('Ctrl Pts',(-20.4166755682946,-16.8710250976204,
-20.5180602073664));
#122787=CARTESIAN_POINT('Ctrl Pts',(-17.8950324982703,-16.4107460543773,
-20.6452360140478));
#122788=CARTESIAN_POINT('Ctrl Pts',(-16.1430851969531,-18.281902167926,
-20.7724118207292));
#122789=CARTESIAN_POINT('Ctrl Pts',(-16.7681507463741,-20.7678461146898,
-20.8995876274106));
#122790=CARTESIAN_POINT('Ctrl Pts',(-19.1967429963892,-21.58783570276,-21.0267634340921));
#122791=CARTESIAN_POINT('Ctrl Pts',(-21.2008319023016,-19.989664067993,
-21.1539392407735));
#122792=CARTESIAN_POINT('Ctrl Pts',(-20.9416889151052,-17.4393951699213,
-21.2811150474549));
#122793=CARTESIAN_POINT('Ctrl Pts',(-18.6572569499448,-16.2770494137143,
-21.4082908541364));
#122794=CARTESIAN_POINT('Ctrl Pts',(-16.4429842219372,-17.568415375407,
-21.5354666608178));
#122795=CARTESIAN_POINT('Ctrl Pts',(-16.3310537276957,-20.1298849908433,
-21.6626424674993));
#122796=CARTESIAN_POINT('Ctrl Pts',(-18.4227563856442,-21.6092689274519,
-21.7898182741806));
#122797=CARTESIAN_POINT('Ctrl Pts',(-20.8017892824853,-20.6535945073695,
-21.9169940808621));
#122798=CARTESIAN_POINT('Ctrl Pts',(-21.2802305760296,-18.1311084332283,
-22.0441698875435));
#122799=CARTESIAN_POINT('Ctrl Pts',(-20.0469417623915,-16.9604786618337,
-22.1289537586645));
#122800=CARTESIAN_POINT('Ctrl Pts',(-19.319022416489,-16.7656980906223,
-22.171345694225));
#122801=CARTESIAN_POINT('Ctrl Pts',(-16.8880688553878,-17.3975534516058,
0.171094837061569));
#122802=CARTESIAN_POINT('Ctrl Pts',(-16.3702697975385,-18.0124051053735,
0.128684244997911));
#122803=CARTESIAN_POINT('Ctrl Pts',(-16.0068254820486,-19.7893209524259,
0.0438817173737748));
#122804=CARTESIAN_POINT('Ctrl Pts',(-17.9658932450075,-21.7021720009294,
-0.0833127458108387));
#122805=CARTESIAN_POINT('Ctrl Pts',(-20.6289595651085,-21.0844926888652,
-0.210488552492274));
#122806=CARTESIAN_POINT('Ctrl Pts',(-21.5536820848537,-18.5139386369225,
-0.337664359173708));
#122807=CARTESIAN_POINT('Ctrl Pts',(-19.8914410613435,-16.3434494886539,
-0.464840165855142));
#122808=CARTESIAN_POINT('Ctrl Pts',(-17.1673608327897,-16.567091225276,
-0.592015972536576));
#122809=CARTESIAN_POINT('Ctrl Pts',(-15.8805535113812,-18.9782470561293,
-0.719191779218011));
#122810=CARTESIAN_POINT('Ctrl Pts',(-17.2116172834215,-21.365578009315,
-0.846367585899445));
#122811=CARTESIAN_POINT('Ctrl Pts',(-19.939366976384,-21.5384685112341,
-0.973543392580879));
#122812=CARTESIAN_POINT('Ctrl Pts',(-21.5612702568039,-19.3385034208011,
-1.10071919926231));
#122813=CARTESIAN_POINT('Ctrl Pts',(-20.5893270128691,-16.7839097584284,
-1.22789500594375));
#122814=CARTESIAN_POINT('Ctrl Pts',(-17.9152371905106,-16.2184228400477,
-1.35507081262518));
#122815=CARTESIAN_POINT('Ctrl Pts',(-15.9923110118271,-18.1608136920126,
-1.48224661930662));
#122816=CARTESIAN_POINT('Ctrl Pts',(-16.5847145272265,-20.8290738621089,
-1.60942242598805));
#122817=CARTESIAN_POINT('Ctrl Pts',(-19.1489539521699,-21.7752326797234,
-1.73659823266948));
#122818=CARTESIAN_POINT('Ctrl Pts',(-21.3324989390857,-20.1312520866371,
-1.86377403935092));
#122819=CARTESIAN_POINT('Ctrl Pts',(-21.1320824002478,-17.4053801994873,
-1.99094984603235));
#122820=CARTESIAN_POINT('Ctrl Pts',(-18.731574116624,-16.0984363471145,
-2.11812565271379));
#122821=CARTESIAN_POINT('Ctrl Pts',(-16.3332914223019,-17.4094598463232,
-2.24530145939522));
#122822=CARTESIAN_POINT('Ctrl Pts',(-16.1375098474575,-20.1356682931634,
-2.37247726607666));
#122823=CARTESIAN_POINT('Ctrl Pts',(-18.3238468290274,-21.7759344971771,
-2.49965307275809));
#122824=CARTESIAN_POINT('Ctrl Pts',(-20.8864738891242,-20.8254160994288,
-2.62682887943953));
#122825=CARTESIAN_POINT('Ctrl Pts',(-21.4743397529562,-18.1561546941444,
-2.75400468612096));
#122826=CARTESIAN_POINT('Ctrl Pts',(-19.5481139784241,-16.2170319683244,
-2.88118049280239));
#122827=CARTESIAN_POINT('Ctrl Pts',(-16.8749891581411,-16.7870726566358,
-3.00835629948383));
#122828=CARTESIAN_POINT('Ctrl Pts',(-15.9073914021204,-19.3432998138438,
-3.13553210616526));
#122829=CARTESIAN_POINT('Ctrl Pts',(-17.533031595496,-21.5405336776668,
-3.2627079128467));
#122830=CARTESIAN_POINT('Ctrl Pts',(-20.2604857595204,-21.3629485552631,
-3.38988371952813));
#122831=CARTESIAN_POINT('Ctrl Pts',(-21.5874839835647,-18.9734677734828,
-3.51705952620957));
#122832=CARTESIAN_POINT('Ctrl Pts',(-20.2965877598843,-16.5642916421105,
-3.644235332891));
#122833=CARTESIAN_POINT('Ctrl Pts',(-17.5721142516412,-16.3456897311358,
-3.77141113957244));
#122834=CARTESIAN_POINT('Ctrl Pts',(-15.9135988027563,-18.5182157260222,
-3.89858694625387));
#122835=CARTESIAN_POINT('Ctrl Pts',(-16.8426263985008,-21.0887118685754,
-4.0257627529353));
#122836=CARTESIAN_POINT('Ctrl Pts',(-19.5068718817363,-21.6989074910159,
-4.15293855961674));
#122837=CARTESIAN_POINT('Ctrl Pts',(-21.4620553833173,-19.7889859827511,
-4.28011436629817));
#122838=CARTESIAN_POINT('Ctrl Pts',(-20.9144173929179,-17.1111817845236,
-4.40729017297961));
#122839=CARTESIAN_POINT('Ctrl Pts',(-18.3663817764822,-16.1222140449305,
-4.53446597966104));
#122840=CARTESIAN_POINT('Ctrl Pts',(-16.1556130631639,-17.7293992827899,
-4.66164178634248));
#122841=CARTESIAN_POINT('Ctrl Pts',(-16.310354331651,-20.4582447955307,
-4.78881759302391));
#122842=CARTESIAN_POINT('Ctrl Pts',(-18.6886400724331,-21.8052041964678,
-4.91599339970535));
#122843=CARTESIAN_POINT('Ctrl Pts',(-21.1085407314031,-20.5345258369701,
-5.04316920638678));
#122844=CARTESIAN_POINT('Ctrl Pts',(-21.34994764993,-17.8119782446832,-5.17034501306821));
#122845=CARTESIAN_POINT('Ctrl Pts',(-19.1913849636685,-16.1353298551694,
-5.29752081974965));
#122846=CARTESIAN_POINT('Ctrl Pts',(-16.6131999617537,-17.0428015012722,
-5.42469662643108));
#122847=CARTESIAN_POINT('Ctrl Pts',(-15.9807173632341,-19.7018442717348,
-5.55187243311253));
#122848=CARTESIAN_POINT('Ctrl Pts',(-17.8742006959542,-21.672951463465,
-5.67904823979394));
#122849=CARTESIAN_POINT('Ctrl Pts',(-20.556496524973,-21.1477545687602,
-5.80622404647539));
#122850=CARTESIAN_POINT('Ctrl Pts',(-21.5667649092206,-18.6080891411163,
-5.93339985315682));
#122851=CARTESIAN_POINT('Ctrl Pts',(-19.9781473104775,-16.3839405809831,
-6.06057565983826));
#122852=CARTESIAN_POINT('Ctrl Pts',(-17.2481017748621,-16.5158271460542,
-6.18775146651969));
#122853=CARTESIAN_POINT('Ctrl Pts',(-15.8812756355658,-18.8827510986805,
-6.31492727320112));
#122854=CARTESIAN_POINT('Ctrl Pts',(-17.1316470405952,-21.3132066201958,
-6.44210307988256));
#122855=CARTESIAN_POINT('Ctrl Pts',(-19.8520778326375,-21.5774016206925,
-6.569278886564));
#122856=CARTESIAN_POINT('Ctrl Pts',(-21.5467416089716,-19.4329535850057,
-6.69645469324542));
#122857=CARTESIAN_POINT('Ctrl Pts',(-20.6608895375072,-16.8472604864224,
-6.82363049992686));
#122858=CARTESIAN_POINT('Ctrl Pts',(-18.0072359116326,-16.1925352566794,
-6.95080630660829));
#122859=CARTESIAN_POINT('Ctrl Pts',(-16.0203432287685,-18.0694476572352,
-7.07798211328973));
#122860=CARTESIAN_POINT('Ctrl Pts',(-16.5230622049748,-20.7560470549016,
-7.20515791997116));
#122861=CARTESIAN_POINT('Ctrl Pts',(-19.0541793818409,-21.7875452514841,
-7.3323337266526));
#122862=CARTESIAN_POINT('Ctrl Pts',(-21.2915518484416,-20.2176066736166,
-7.45950953333402));
#122863=CARTESIAN_POINT('Ctrl Pts',(-21.1825292336674,-17.4865525251151,
-7.58668534001548));
#122864=CARTESIAN_POINT('Ctrl Pts',(-18.8271330198668,-16.0999554788923,
-7.71386114669689));
#122865=CARTESIAN_POINT('Ctrl Pts',(-16.3862930408257,-17.3299322629389,
-7.84103695337835));
#122866=CARTESIAN_POINT('Ctrl Pts',(-16.0993284816994,-20.0480555188611,
-7.96821276005976));
#122867=CARTESIAN_POINT('Ctrl Pts',(-18.2295115144572,-21.760615865106,
-8.09538856674121));
#122868=CARTESIAN_POINT('Ctrl Pts',(-20.8225314206137,-20.8964454774766,
-8.22256437342263));
#122869=CARTESIAN_POINT('Ctrl Pts',(-21.4994533772365,-18.2483670501596,
-8.34974018010408));
#122870=CARTESIAN_POINT('Ctrl Pts',(-19.6392435036391,-16.245828181935,
-8.4769159867855));
#122871=CARTESIAN_POINT('Ctrl Pts',(-16.9485289012012,-16.7260339928192,
-8.60409179346695));
#122872=CARTESIAN_POINT('Ctrl Pts',(-15.8958732130767,-19.2484254562599,
-8.73126760014836));
#122873=CARTESIAN_POINT('Ctrl Pts',(-17.4470226979395,-21.4988649618209,
-8.85844340682981));
#122874=CARTESIAN_POINT('Ctrl Pts',(-20.1788939786226,-21.4127139411785,
-8.98561921351124));
#122875=CARTESIAN_POINT('Ctrl Pts',(-21.5851647141539,-19.0690106086366,
-9.11279502019268));
#122876=CARTESIAN_POINT('Ctrl Pts',(-20.3756687876888,-16.617957305168,
-9.23997082687412));
#122877=CARTESIAN_POINT('Ctrl Pts',(-17.6600436419756,-16.3082433071803,
-9.36714663355554));
#122878=CARTESIAN_POINT('Ctrl Pts',(-15.9297067975006,-18.4240119848083,
-9.49432244023699));
#122879=CARTESIAN_POINT('Ctrl Pts',(-16.772134912253,-21.0241768957426,
-9.62149824691841));
#122880=CARTESIAN_POINT('Ctrl Pts',(-19.4144524779331,-21.7232481186362,
-9.74867405359986));
#122881=CARTESIAN_POINT('Ctrl Pts',(-21.4324971287534,-19.8798711957376,
-9.87584986028127));
#122882=CARTESIAN_POINT('Ctrl Pts',(-20.9748381515633,-17.1852300409311,
-10.0030256669627));
#122883=CARTESIAN_POINT('Ctrl Pts',(-18.461349252415,-16.1114906654595,
-10.1302014736441));
#122884=CARTESIAN_POINT('Ctrl Pts',(-16.1980004915621,-17.6437423025364,
-10.2573772803256));
#122885=CARTESIAN_POINT('Ctrl Pts',(-16.2612738778198,-20.3762391774058,
-10.384553087007));
#122886=CARTESIAN_POINT('Ctrl Pts',(-18.5931200064859,-21.8020850052583,
-10.5117288936884));
#122887=CARTESIAN_POINT('Ctrl Pts',(-21.0542147852026,-20.6131547370118,
-10.6389047003698));
#122888=CARTESIAN_POINT('Ctrl Pts',(-21.3866565072667,-17.900218100448,
-10.7660805070513));
#122889=CARTESIAN_POINT('Ctrl Pts',(-19.2854505263445,-16.152226075776,
-10.8932563137327));
#122890=CARTESIAN_POINT('Ctrl Pts',(-16.6783229143809,-16.9728528530119,
-11.0204321204142));
#122891=CARTESIAN_POINT('Ctrl Pts',(-15.9571514387634,-19.6092242978837,
-11.1476079270956));
#122892=CARTESIAN_POINT('Ctrl Pts',(-17.7835661674212,-21.6426332413875,
-11.274783733777));
#122893=CARTESIAN_POINT('Ctrl Pts',(-20.4819449468934,-21.2075531854514,
-11.4019595404585));
#122894=CARTESIAN_POINT('Ctrl Pts',(-21.5766927272896,-18.7031430772827,
-11.5291353471399));
#122895=CARTESIAN_POINT('Ctrl Pts',(-20.0634463678067,-16.4270437499047,
-11.6563111538213));
#122896=CARTESIAN_POINT('Ctrl Pts',(-17.3305154806086,-16.4674350655298,
-11.7834869605028));
#122897=CARTESIAN_POINT('Ctrl Pts',(-15.8851945298786,-18.78726049904,-11.9106627671842));
#122898=CARTESIAN_POINT('Ctrl Pts',(-17.0534757811762,-21.2582241997943,
-12.0378385738656));
#122899=CARTESIAN_POINT('Ctrl Pts',(-19.7635336981482,-21.6133703376545,
-12.1650143805471));
#122900=CARTESIAN_POINT('Ctrl Pts',(-21.5290583471371,-19.526874373989,
-12.2921901872285));
#122901=CARTESIAN_POINT('Ctrl Pts',(-20.7302904435137,-16.9129668529163,
-12.4193659939099));
#122902=CARTESIAN_POINT('Ctrl Pts',(-18.1000499617251,-16.1697456876228,
-12.5465418005913));
#122903=CARTESIAN_POINT('Ctrl Pts',(-16.0514192926768,-17.9790701677574,
-12.6737176072728));
#122904=CARTESIAN_POINT('Ctrl Pts',(-16.4638899228612,-20.6809973821388,
-12.8008934139542));
#122905=CARTESIAN_POINT('Ctrl Pts',(-18.9590456498985,-21.7966768120881,
-12.9280692206357));
#122906=CARTESIAN_POINT('Ctrl Pts',(-21.2477359610623,-20.3025418275019,
-13.0552450273171));
#122907=CARTESIAN_POINT('Ctrl Pts',(-21.2302295480009,-17.569368540262,
-13.1824208339985));
#122908=CARTESIAN_POINT('Ctrl Pts',(-18.9225874581277,-16.1046738015453,
-13.30959664068));
#122909=CARTESIAN_POINT('Ctrl Pts',(-16.44192808048,-17.2522241249159,-13.4367724473614));
#122910=CARTESIAN_POINT('Ctrl Pts',(-16.0641024269644,-19.9592133136872,
-13.5639482540428));
#122911=CARTESIAN_POINT('Ctrl Pts',(-18.1357420841767,-21.7421468018591,
-13.6911240607243));
#122912=CARTESIAN_POINT('Ctrl Pts',(-20.7562462470829,-20.9652937753664,
-13.8182998674057));
#122913=CARTESIAN_POINT('Ctrl Pts',(-21.521464993048,-18.3413686690794,
-13.9454756740872));
#122914=CARTESIAN_POINT('Ctrl Pts',(-19.7293576174809,-16.2776599088574,
-14.0726514807686));
#122915=CARTESIAN_POINT('Ctrl Pts',(-17.0240714067361,-16.6674921939926,
-14.19982728745));
#122916=CARTESIAN_POINT('Ctrl Pts',(-15.8875385501732,-19.1532185985939,
-14.3270030941314));
#122917=CARTESIAN_POINT('Ctrl Pts',(-17.3624574025039,-21.4543394280201,
-14.4541789008129));
#122918=CARTESIAN_POINT('Ctrl Pts',(-20.0956814605031,-21.4597191449386,
-14.5813547074943));
#122919=CARTESIAN_POINT('Ctrl Pts',(-21.5796472939737,-19.1644221929799,
-14.7085305141757));
#122920=CARTESIAN_POINT('Ctrl Pts',(-20.4529083560135,-16.6742410633702,
-14.8357063208572));
#122921=CARTESIAN_POINT('Ctrl Pts',(-17.7491776888957,-16.2737623844548,
-14.9628821275386));
#122922=CARTESIAN_POINT('Ctrl Pts',(-15.9489603672498,-18.3304004876284,
-15.0900579342201));
#122923=CARTESIAN_POINT('Ctrl Pts',(-16.7038440495977,-20.9573175625861,
-15.2172337409015));
#122924=CARTESIAN_POINT('Ctrl Pts',(-19.3212698107507,-21.7444802379159,
-15.3444095475829));
#122925=CARTESIAN_POINT('Ctrl Pts',(-21.3999119706151,-19.9697156158284,
-15.4715853542643));
#122926=CARTESIAN_POINT('Ctrl Pts',(-21.032745362598,-17.2612600827733,
-15.5987611609458));
#122927=CARTESIAN_POINT('Ctrl Pts',(-18.5566225606254,-16.1039534846195,
-15.7259369676272));
#122928=CARTESIAN_POINT('Ctrl Pts',(-16.2432325499933,-17.5595527946246,
-15.8531127743086));
#122929=CARTESIAN_POINT('Ctrl Pts',(-16.2149670802795,-20.2926359905412,
-15.9802885809901));
#122930=CARTESIAN_POINT('Ctrl Pts',(-18.4977579655933,-21.7957688743899,
-16.1074643876715));
#122931=CARTESIAN_POINT('Ctrl Pts',(-20.997286254641,-20.6899203201883,
-16.234640194353));
#122932=CARTESIAN_POINT('Ctrl Pts',(-21.4203898804431,-17.9896377397141,
-16.3618160010344));
#122933=CARTESIAN_POINT('Ctrl Pts',(-19.378897527099,-16.1722628021139,
-16.4889918077158));
#122934=CARTESIAN_POINT('Ctrl Pts',(-16.7457517194962,-16.9051242136259,
-16.6161676143973));
#122935=CARTESIAN_POINT('Ctrl Pts',(-15.9367003046499,-19.5158671156972,
-16.7433434210787));
#122936=CARTESIAN_POINT('Ctrl Pts',(-17.6939977402874,-21.6092969366562,
-16.8705192277601));
#122937=CARTESIAN_POINT('Ctrl Pts',(-20.4054326993911,-21.2648217486819,
-16.9976950344416));
#122938=CARTESIAN_POINT('Ctrl Pts',(-21.5834318976165,-18.798476156199,
-17.124870841123));
#122939=CARTESIAN_POINT('Ctrl Pts',(-20.147254185468,-16.4729791616393,
-17.2520466478045));
#122940=CARTESIAN_POINT('Ctrl Pts',(-17.4145034745997,-16.4218299208892,
-17.3792224544858));
#122941=CARTESIAN_POINT('Ctrl Pts',(-15.8923089285959,-18.691954687658,
-17.5063982611673));
#122942=CARTESIAN_POINT('Ctrl Pts',(-16.9771895653652,-21.200654888267,
-17.6335740678487));
#122943=CARTESIAN_POINT('Ctrl Pts',(-19.6738347359604,-21.646353796156,
-17.7607498745302));
#122944=CARTESIAN_POINT('Ctrl Pts',(-21.5082398690315,-19.6201503265241,
-17.8879256812116));
#122945=CARTESIAN_POINT('Ctrl Pts',(-20.7974521110171,-16.980960402401,
-18.015101487893));
#122946=CARTESIAN_POINT('Ctrl Pts',(-18.1935751134159,-16.1500769725442,
-18.1422772945745));
#122947=CARTESIAN_POINT('Ctrl Pts',(-16.0855044067243,-17.8897840134535,
-18.2694531012559));
#122948=CARTESIAN_POINT('Ctrl Pts',(-16.407264022649,-20.6040082933991,
-18.3966289079374));
#122949=CARTESIAN_POINT('Ctrl Pts',(-18.8636594843459,-21.8026174994663,
-18.5238047146188));
#122950=CARTESIAN_POINT('Ctrl Pts',(-21.2011004165875,-20.3859620788242,
-18.6509805213002));
#122951=CARTESIAN_POINT('Ctrl Pts',(-21.275129842407,-17.6537354530185,
-18.7781563279817));
#122952=CARTESIAN_POINT('Ctrl Pts',(-19.0178303575923,-16.1125859688478,
-18.9053321346631));
#122953=CARTESIAN_POINT('Ctrl Pts',(-16.500134137209,-17.1764226259579,
-19.0325079413445));
#122954=CARTESIAN_POINT('Ctrl Pts',(-16.031871194612,-19.8692413158911,
-19.1596837480259));
#122955=CARTESIAN_POINT('Ctrl Pts',(-18.0426437217303,-21.7205480348836,
-19.2868595547074));
#122956=CARTESIAN_POINT('Ctrl Pts',(-20.6876927164292,-21.0318837558328,
-19.4140353613888));
#122957=CARTESIAN_POINT('Ctrl Pts',(-21.5403499177572,-18.4350552451234,
-19.5412111680702));
#122958=CARTESIAN_POINT('Ctrl Pts',(-19.8183552240814,-16.3124914190809,
-19.6683869747517));
#122959=CARTESIAN_POINT('Ctrl Pts',(-17.1015319673585,-16.6115129719686,
-19.7955627814331));
#122960=CARTESIAN_POINT('Ctrl Pts',(-15.8823967072827,-19.0577859474646,
-19.9227385881146));
#122961=CARTESIAN_POINT('Ctrl Pts',(-17.2794306722399,-21.4070071875673,
-20.049914394796));
#122962=CARTESIAN_POINT('Ctrl Pts',(-20.0109413400502,-21.5039111192106,
-20.1770902014774));
#122963=CARTESIAN_POINT('Ctrl Pts',(-21.5709383060712,-19.2595961229167,
-20.3042660081589));
#122964=CARTESIAN_POINT('Ctrl Pts',(-20.5282190658065,-16.7330785895595,
-20.4314418148403));
#122965=CARTESIAN_POINT('Ctrl Pts',(-17.8394178740343,-16.242287940109,
-20.5586176215217));
#122966=CARTESIAN_POINT('Ctrl Pts',(-15.9713350959043,-18.2374818071192,
-20.6857934282032));
#122967=CARTESIAN_POINT('Ctrl Pts',(-16.6378358446413,-20.8882174033637,
-20.8129692348846));
#122968=CARTESIAN_POINT('Ctrl Pts',(-19.2274179364899,-21.762563581795,
-20.9401450415661));
#122969=CARTESIAN_POINT('Ctrl Pts',(-21.3643566264617,-20.0584501617399,
-21.0673208482474));
#122970=CARTESIAN_POINT('Ctrl Pts',(-21.0880352148013,-17.3391255539126,
-21.1944966549289));
#122971=CARTESIAN_POINT('Ctrl Pts',(-18.6521697017704,-16.099728633828,
-21.3216724616103));
#122972=CARTESIAN_POINT('Ctrl Pts',(-16.2911142372801,-17.4766984270906,
-21.4488482682919));
#122973=CARTESIAN_POINT('Ctrl Pts',(-16.171763941479,-20.2079662407414,
-21.5760240749732));
#122974=CARTESIAN_POINT('Ctrl Pts',(-18.4021242436095,-21.7854176013747,
-21.7031998816546));
#122975=CARTESIAN_POINT('Ctrl Pts',(-20.9388617241559,-20.7663921293681,
-21.8303756883361));
#122976=CARTESIAN_POINT('Ctrl Pts',(-21.4490185879752,-18.0766920512704,
-21.9575514950175));
#122977=CARTESIAN_POINT('Ctrl Pts',(-20.1339758401221,-16.8284619738791,
-22.0423353661385));
#122978=CARTESIAN_POINT('Ctrl Pts',(-19.3578031818887,-16.6207695219882,
-22.0847273016989));
#122979=CARTESIAN_POINT('Ctrl Pts',(-16.7733105073354,-17.3009161969877,
0.257713229587529));
#122980=CARTESIAN_POINT('Ctrl Pts',(-16.2233207772202,-17.9539921151271,
0.215302637523872));
#122981=CARTESIAN_POINT('Ctrl Pts',(-15.8372817569514,-19.8413757484949,
0.130500109899736));
#122982=CARTESIAN_POINT('Ctrl Pts',(-17.9181413759371,-21.8731454397858,
0.00330564671512246));
#122983=CARTESIAN_POINT('Ctrl Pts',(-20.7467659253037,-21.217066072722,
-0.123870159966312));
#122984=CARTESIAN_POINT('Ctrl Pts',(-21.7289768454601,-18.4867051192915,
-0.251045966647746));
#122985=CARTESIAN_POINT('Ctrl Pts',(-19.9633971711666,-16.1812804129726,
-0.378221773329182));
#122986=CARTESIAN_POINT('Ctrl Pts',(-17.0699655841381,-16.4188255697332,
-0.505397580010615));
#122987=CARTESIAN_POINT('Ctrl Pts',(-15.703159676164,-18.9798787902334,
-0.632573386692051));
#122988=CARTESIAN_POINT('Ctrl Pts',(-17.1169733817962,-21.5156259816095,
-0.759749193373484));
#122989=CARTESIAN_POINT('Ctrl Pts',(-20.0143025574919,-21.6992647871434,
-0.886925000054919));
#122990=CARTESIAN_POINT('Ctrl Pts',(-21.737036760942,-19.362531670293,-1.01410080673635));
#122991=CARTESIAN_POINT('Ctrl Pts',(-20.7046694858076,-16.6491233362602,
-1.14127661341778));
#122992=CARTESIAN_POINT('Ctrl Pts',(-17.8643361221052,-16.0484810737661,
-1.26845242009922));
#122993=CARTESIAN_POINT('Ctrl Pts',(-15.8218649472086,-18.1116270070318,
-1.39562822678065));
#122994=CARTESIAN_POINT('Ctrl Pts',(-16.4510971650251,-20.9457682990692,
-1.52280403346208));
#122995=CARTESIAN_POINT('Ctrl Pts',(-19.1747509220124,-21.9507481746746,
-1.64997984014352));
#122996=CARTESIAN_POINT('Ctrl Pts',(-21.4940431258966,-20.2045641501962,
-1.77715564682495));
#122997=CARTESIAN_POINT('Ctrl Pts',(-21.2811670373152,-17.3092295202543,
-1.90433145350639));
#122998=CARTESIAN_POINT('Ctrl Pts',(-18.7314233036483,-15.9210352279973,
-2.03150726018783));
#122999=CARTESIAN_POINT('Ctrl Pts',(-16.1840435203226,-17.3135627916812,
-2.15868306686926));
#123000=CARTESIAN_POINT('Ctrl Pts',(-15.9760905434333,-20.2092549046476,
-2.28585887355069));
#123001=CARTESIAN_POINT('Ctrl Pts',(-18.2983483154525,-21.9514936229061,
-2.41303468023213));
#123002=CARTESIAN_POINT('Ctrl Pts',(-21.020289469658,-20.9418831396066,
-2.54021048691356));
#123003=CARTESIAN_POINT('Ctrl Pts',(-21.644701937954,-18.1066783673205,
-2.66738629359499));
#123004=CARTESIAN_POINT('Ctrl Pts',(-19.598726037039,-16.0470037339522,
-2.79456210027643));
#123005=CARTESIAN_POINT('Ctrl Pts',(-16.7594176679228,-16.6524828663812,
-2.92173790695786));
#123006=CARTESIAN_POINT('Ctrl Pts',(-15.7316660321737,-19.3676262467993,
-3.0489137136393));
#123007=CARTESIAN_POINT('Ctrl Pts',(-17.4583694659978,-21.701458341403,
-3.17608952032073));
#123008=CARTESIAN_POINT('Ctrl Pts',(-20.3553847402323,-21.512833058945,
-3.30326532700217));
#123009=CARTESIAN_POINT('Ctrl Pts',(-21.7648801497778,-18.9748023878472,
-3.4304411336836));
#123010=CARTESIAN_POINT('Ctrl Pts',(-20.3937311395464,-16.4158519413221,
-3.55761694036504));
#123011=CARTESIAN_POINT('Ctrl Pts',(-17.4998818233102,-16.1836599274567,
-3.68479274704647));
#123012=CARTESIAN_POINT('Ctrl Pts',(-15.7382593361759,-18.4912481076264,
-3.8119685537279));
#123013=CARTESIAN_POINT('Ctrl Pts',(-16.7250429714639,-21.2215475515407,
-3.93914436040934));
#123014=CARTESIAN_POINT('Ctrl Pts',(-19.5549199904986,-21.8696779809346,
-4.06632016709077));
#123015=CARTESIAN_POINT('Ctrl Pts',(-21.6316538702915,-19.8410199543343,
-4.19349597377222));
#123016=CARTESIAN_POINT('Ctrl Pts',(-21.0499701727744,-16.9967412984365,
-4.32067178045365));
#123017=CARTESIAN_POINT('Ctrl Pts',(-18.3435275870569,-15.9462911441802,
-4.44784758713508));
#123018=CARTESIAN_POINT('Ctrl Pts',(-15.9953192047637,-17.6533923098082,
-4.57502339381652));
#123019=CARTESIAN_POINT('Ctrl Pts',(-16.159680470399,-20.5518854305035,
-4.70219920049796));
#123020=CARTESIAN_POINT('Ctrl Pts',(-18.6858201241535,-21.9825829688008,
-4.82937500717938));
#123021=CARTESIAN_POINT('Ctrl Pts',(-21.2561618236167,-20.6329087324161,
-4.95655081386081));
#123022=CARTESIAN_POINT('Ctrl Pts',(-21.5125765929291,-17.7411050630016,
-5.08372662054226));
#123023=CARTESIAN_POINT('Ctrl Pts',(-19.219819796142,-15.9602223416674,
-5.21090242722368));
#123024=CARTESIAN_POINT('Ctrl Pts',(-16.4813534897718,-16.9241099311898,
-5.33807823390512));
#123025=CARTESIAN_POINT('Ctrl Pts',(-15.8095505415254,-19.748460793793,
-5.46525404058655));
#123026=CARTESIAN_POINT('Ctrl Pts',(-17.8207484596252,-21.8421083120231,
-5.59242984726799));
#123027=CARTESIAN_POINT('Ctrl Pts',(-20.6697979832357,-21.2842608343242,
-5.71960565394942));
#123028=CARTESIAN_POINT('Ctrl Pts',(-21.7428730064005,-18.5867087975656,
-5.84678146063087));
#123029=CARTESIAN_POINT('Ctrl Pts',(-20.0554937979133,-16.2242887665116,
-5.9739572673123));
#123030=CARTESIAN_POINT('Ctrl Pts',(-17.1557260509959,-16.3643744913304,
-6.10113307399374));
#123031=CARTESIAN_POINT('Ctrl Pts',(-15.7039266935608,-18.8784460142016,
-6.22830888067515));
#123032=CARTESIAN_POINT('Ctrl Pts',(-17.0320315272241,-21.4599987537674,
-6.35548468735659));
#123033=CARTESIAN_POINT('Ctrl Pts',(-19.9215867985823,-21.7406183007101,
-6.48266049403803));
#123034=CARTESIAN_POINT('Ctrl Pts',(-21.7216048921908,-19.4628536379228,
-6.60983630071946));
#123035=CARTESIAN_POINT('Ctrl Pts',(-20.7806809288866,-16.7164124694941,
-6.73701210740091));
#123036=CARTESIAN_POINT('Ctrl Pts',(-17.9620542446739,-16.0209841040936,
-6.86418791408233));
#123037=CARTESIAN_POINT('Ctrl Pts',(-15.8516398786156,-18.0145809038241,
-6.99136372076378));
#123038=CARTESIAN_POINT('Ctrl Pts',(-16.3856120244824,-20.868201541505,
-7.1185395274452));
#123039=CARTESIAN_POINT('Ctrl Pts',(-19.0740843804904,-21.9638261977359,
-7.24571533412664));
#123040=CARTESIAN_POINT('Ctrl Pts',(-21.4505504254156,-20.2962872525602,
-7.37289114080807));
#123041=CARTESIAN_POINT('Ctrl Pts',(-21.3347500631569,-17.3954481890373,
-7.50006694748951));
#123042=CARTESIAN_POINT('Ctrl Pts',(-18.8329229387055,-15.9226488015715,
-7.62724275417095));
#123043=CARTESIAN_POINT('Ctrl Pts',(-16.2403401578418,-17.2290911159235,
-7.75441856085238));
#123044=CARTESIAN_POINT('Ctrl Pts',(-15.9355355081732,-20.1161953956302,
-7.8815943675338));
#123045=CARTESIAN_POINT('Ctrl Pts',(-18.1981483374604,-21.9352226579616,
-8.00877017421523));
#123046=CARTESIAN_POINT('Ctrl Pts',(-20.9523718084227,-21.0173282912935,
-8.13594598089667));
#123047=CARTESIAN_POINT('Ctrl Pts',(-21.6713768328398,-18.2046234060944,
-8.26312178757811));
#123048=CARTESIAN_POINT('Ctrl Pts',(-19.6955209272938,-16.0775901583807,
-8.39029759425955));
#123049=CARTESIAN_POINT('Ctrl Pts',(-16.837529249675,-16.5876495343575,
-8.51747340094098));
#123050=CARTESIAN_POINT('Ctrl Pts',(-15.7194317772296,-19.2668537144213,
-8.64464920762241));
#123051=CARTESIAN_POINT('Ctrl Pts',(-17.3670135439705,-21.657199153529,
-8.77182501430385));
#123052=CARTESIAN_POINT('Ctrl Pts',(-20.2687205393704,-21.5656922728693,
-8.89900082098528));
#123053=CARTESIAN_POINT('Ctrl Pts',(-21.7624166953973,-19.07628495589,-9.02617662766673));
#123054=CARTESIAN_POINT('Ctrl Pts',(-20.4777284981358,-16.4728539058758,
-9.15335243434816));
#123055=CARTESIAN_POINT('Ctrl Pts',(-17.5932776318311,-16.1438855240604,
-9.28052824102959));
#123056=CARTESIAN_POINT('Ctrl Pts',(-15.7553687371063,-18.3911878826788,
-9.40770404771103));
#123057=CARTESIAN_POINT('Ctrl Pts',(-16.6501691513803,-21.1530005510137,
-9.53487985439245));
#123058=CARTESIAN_POINT('Ctrl Pts',(-19.4567550321338,-21.8955318232944,
-9.6620556610739));
#123059=CARTESIAN_POINT('Ctrl Pts',(-21.6002580301411,-19.9375553438918,
-9.78923146775533));
#123060=CARTESIAN_POINT('Ctrl Pts',(-21.1141471855306,-17.0753930069318,
-9.91640727443676));
#123061=CARTESIAN_POINT('Ctrl Pts',(-18.4443990267908,-15.9349011107458,
-10.0435830811182));
#123062=CARTESIAN_POINT('Ctrl Pts',(-16.0403417863069,-17.5624101831744,
-10.1707588877996));
#123063=CARTESIAN_POINT('Ctrl Pts',(-16.1075487696024,-20.4647816648694,
-10.297934694481));
#123064=CARTESIAN_POINT('Ctrl Pts',(-18.5843617408396,-21.9792698628662,
-10.4251105011625));
#123065=CARTESIAN_POINT('Ctrl Pts',(-21.1984585272586,-20.7164258552413,
-10.5522863078439));
#123066=CARTESIAN_POINT('Ctrl Pts',(-21.5515675764649,-17.8348306380519,
-10.6794621145253));
#123067=CARTESIAN_POINT('Ctrl Pts',(-19.319733252231,-15.9781689710992,
-10.8066379212068));
#123068=CARTESIAN_POINT('Ctrl Pts',(-16.5505250237807,-16.849812696393,
-10.9338137278882));
#123069=CARTESIAN_POINT('Ctrl Pts',(-15.7845195642707,-19.6500827962871,
-11.0609895345697));
#123070=CARTESIAN_POINT('Ctrl Pts',(-17.7244793391404,-21.8099052584926,
-11.1881653412511));
#123071=CARTESIAN_POINT('Ctrl Pts',(-20.5906116624301,-21.3477770276364,
-11.3153411479325));
#123072=CARTESIAN_POINT('Ctrl Pts',(-21.753418019756,-18.6876720726163,
-11.442516954614));
#123073=CARTESIAN_POINT('Ctrl Pts',(-20.1460957501734,-16.2700715849292,
-11.5696927612954));
#123074=CARTESIAN_POINT('Ctrl Pts',(-17.2432632743535,-16.3129739588191,
-11.6968685679768));
#123075=CARTESIAN_POINT('Ctrl Pts',(-15.7080892187581,-18.7770189290635,
-11.8240443746583));
#123076=CARTESIAN_POINT('Ctrl Pts',(-16.9490004957481,-21.4015981713421,
-11.9512201813397));
#123077=CARTESIAN_POINT('Ctrl Pts',(-19.8275380283252,-21.7788231306235,
-12.0783959880211));
#123078=CARTESIAN_POINT('Ctrl Pts',(-21.7028222925386,-19.5626133199888,
-12.2055717947026));
#123079=CARTESIAN_POINT('Ctrl Pts',(-20.8543963692405,-16.7862036872011,
-12.332747601384));
#123080=CARTESIAN_POINT('Ctrl Pts',(-18.0606383838055,-15.996777746927,
-12.4599234080654));
#123081=CARTESIAN_POINT('Ctrl Pts',(-15.8846478876935,-17.9185848020682,
-12.5870992147468));
#123082=CARTESIAN_POINT('Ctrl Pts',(-16.3227611038855,-20.7884861603309,
-12.7142750214283));
#123083=CARTESIAN_POINT('Ctrl Pts',(-18.9730363488984,-21.9735254516762,
-12.8414508281097));
#123084=CARTESIAN_POINT('Ctrl Pts',(-21.404010580066,-20.3865026781285,
-12.9686266347912));
#123085=CARTESIAN_POINT('Ctrl Pts',(-21.3854158235693,-17.4834127326752,
-13.0958024414726));
#123086=CARTESIAN_POINT('Ctrl Pts',(-18.9343116143732,-15.9276604541869,
-13.222978248154));
#123087=CARTESIAN_POINT('Ctrl Pts',(-16.2994339317307,-17.1465519972999,
-13.3501540548355));
#123088=CARTESIAN_POINT('Ctrl Pts',(-15.8981195105134,-20.0218300241493,
-13.4773298615169));
#123089=CARTESIAN_POINT('Ctrl Pts',(-18.0985494238061,-21.9156054049817,
-13.6045056681983));
#123090=CARTESIAN_POINT('Ctrl Pts',(-20.8819658002459,-21.0904567688396,
-13.7316814748798));
#123091=CARTESIAN_POINT('Ctrl Pts',(-21.694756872753,-18.3034067748831,
-13.8588572815612));
#123092=CARTESIAN_POINT('Ctrl Pts',(-19.7912372798057,-16.1114008087357,
-13.9860330882426));
#123093=CARTESIAN_POINT('Ctrl Pts',(-16.9177681021827,-16.5254682931038,
-14.1132088949241));
#123094=CARTESIAN_POINT('Ctrl Pts',(-15.7105789627421,-19.1657280110059,
-14.2403847016055));
#123095=CARTESIAN_POINT('Ctrl Pts',(-17.2771909703125,-21.6099055442666,
-14.367560508287));
#123096=CARTESIAN_POINT('Ctrl Pts',(-20.1803348428554,-21.6156197088857,
-14.4947363149684));
#123097=CARTESIAN_POINT('Ctrl Pts',(-21.7565562667429,-19.1776281134862,
-14.6219121216498));
#123098=CARTESIAN_POINT('Ctrl Pts',(-20.5597699168931,-16.5326367280232,
-14.7490879283312));
#123099=CARTESIAN_POINT('Ctrl Pts',(-17.6879529883551,-16.107260981979,
-14.8762637350127));
#123100=CARTESIAN_POINT('Ctrl Pts',(-15.7758192680016,-18.2917567205529,
-15.0034395416941));
#123101=CARTESIAN_POINT('Ctrl Pts',(-16.5776327638535,-21.0819846886999,
-15.1306153483755));
#123102=CARTESIAN_POINT('Ctrl Pts',(-19.3577793596249,-21.9180839067241,
-15.257791155057));
#123103=CARTESIAN_POINT('Ctrl Pts',(-21.5656471090539,-20.0329852362584,
-15.3849669617384));
#123104=CARTESIAN_POINT('Ctrl Pts',(-21.1756543877665,-17.1561497050361,
-15.5121427684199));
#123105=CARTESIAN_POINT('Ctrl Pts',(-18.545595311866,-15.9268953564031,
-15.6393185751013));
#123106=CARTESIAN_POINT('Ctrl Pts',(-16.0883858436145,-17.4729867591009,
-15.7664943817827));
#123107=CARTESIAN_POINT('Ctrl Pts',(-16.0583631585132,-20.3759810124089,
-15.8936701884641));
#123108=CARTESIAN_POINT('Ctrl Pts',(-18.4830712067246,-21.9725610690611,
-16.0208459951456));
#123109=CARTESIAN_POINT('Ctrl Pts',(-21.1379908483687,-20.7979638220132,
-16.148021801827));
#123110=CARTESIAN_POINT('Ctrl Pts',(-21.5873980951341,-17.9298093417044,
-16.2751976085084));
#123111=CARTESIAN_POINT('Ctrl Pts',(-19.418989691473,-15.9994513460744,
-16.4023734151899));
#123112=CARTESIAN_POINT('Ctrl Pts',(-16.6221457611405,-16.7778734845843,
-16.5295492218713));
#123113=CARTESIAN_POINT('Ctrl Pts',(-15.7627970185048,-19.550921759478,
-16.6567250285528));
#123114=CARTESIAN_POINT('Ctrl Pts',(-17.6293425977359,-21.7744964933273,
-16.7839008352342));
#123115=CARTESIAN_POINT('Ctrl Pts',(-20.5093427807734,-21.4086058784384,
-16.9110766419156));
#123116=CARTESIAN_POINT('Ctrl Pts',(-21.7605761526514,-18.7889318442388,
-17.0382524485971));
#123117=CARTESIAN_POINT('Ctrl Pts',(-20.2351137549734,-16.3188627217991,
-17.1654282552785));
#123118=CARTESIAN_POINT('Ctrl Pts',(-17.3324726567343,-16.2645336211774,
-17.2926040619599));
#123119=CARTESIAN_POINT('Ctrl Pts',(-15.7156459073444,-18.6757881201507,
-17.4197798686414));
#123120=CARTESIAN_POINT('Ctrl Pts',(-16.8679716977821,-21.3404498752418,
-17.5469556753228));
#123121=CARTESIAN_POINT('Ctrl Pts',(-19.7322626367279,-21.813857113719,
-17.6741314820042));
#123122=CARTESIAN_POINT('Ctrl Pts',(-21.6807095656397,-19.6616880772395,
-17.8013072886857));
#123123=CARTESIAN_POINT('Ctrl Pts',(-20.925733361505,-16.8584242781114,
-17.9284830953671));
#123124=CARTESIAN_POINT('Ctrl Pts',(-18.1599778324925,-15.9758862618349,
-18.0556589020486));
#123125=CARTESIAN_POINT('Ctrl Pts',(-15.9208520143557,-17.8237478819072,
-18.18283470873));
#123126=CARTESIAN_POINT('Ctrl Pts',(-16.2626148693509,-20.7067107930414,
-18.3100105154114));
#123127=CARTESIAN_POINT('Ctrl Pts',(-18.871720190335,-21.9798354613185,
-18.4371863220928));
#123128=CARTESIAN_POINT('Ctrl Pts',(-21.3544757844137,-20.4751090222602,
-18.5643621287743));
#123129=CARTESIAN_POINT('Ctrl Pts',(-21.4331074916559,-17.573024590546,
-18.6915379354557));
#123130=CARTESIAN_POINT('Ctrl Pts',(-19.0354756002437,-15.9360645072522,
-18.8187137421372));
#123131=CARTESIAN_POINT('Ctrl Pts',(-16.3612585583812,-17.0660380501958,
-18.9458895488186));
#123132=CARTESIAN_POINT('Ctrl Pts',(-15.8638845181663,-19.926264622792,
-19.0730653555));
#123133=CARTESIAN_POINT('Ctrl Pts',(-17.9996632971129,-21.8926638800028,
-19.2002411621814));
#123134=CARTESIAN_POINT('Ctrl Pts',(-20.8091504151054,-21.1611865332722,
-19.3274169688629));
#123135=CARTESIAN_POINT('Ctrl Pts',(-21.7148158405836,-18.4029176833963,
-19.4545927755443));
#123136=CARTESIAN_POINT('Ctrl Pts',(-19.8857677137514,-16.1483977337339,
-19.5817685822257));
#123137=CARTESIAN_POINT('Ctrl Pts',(-17.0000442519466,-16.4660089396223,
-19.7089443889072));
#123138=CARTESIAN_POINT('Ctrl Pts',(-15.7051174603682,-19.0643624769379,
-19.8361201955886));
#123139=CARTESIAN_POINT('Ctrl Pts',(-17.1890026117629,-21.5596307402518,
-19.9632960022701));
#123140=CARTESIAN_POINT('Ctrl Pts',(-20.0903265756109,-21.6625590217998,
-20.0904718089515));
#123141=CARTESIAN_POINT('Ctrl Pts',(-21.7473058561185,-19.2787188421125,
-20.2176476156329));
#123142=CARTESIAN_POINT('Ctrl Pts',(-20.6397625633182,-16.5951320814986,
-20.3448234223144));
#123143=CARTESIAN_POINT('Ctrl Pts',(-17.7838032497984,-16.0738298258407,
-20.4719992289958));
#123144=CARTESIAN_POINT('Ctrl Pts',(-15.7995849948555,-18.1930614463123,
-20.5991750356772));
#123145=CARTESIAN_POINT('Ctrl Pts',(-16.5075209429087,-21.0085886920376,
-20.7263508423587));
#123146=CARTESIAN_POINT('Ctrl Pts',(-19.2580928765906,-21.9372914608301,
-20.8535266490401));
#123147=CARTESIAN_POINT('Ctrl Pts',(-21.5278813506218,-20.1272362554868,
-20.9807024557215));
#123148=CARTESIAN_POINT('Ctrl Pts',(-21.2343815144973,-17.2388559379038,
-21.107878262403));
#123149=CARTESIAN_POINT('Ctrl Pts',(-18.647082453596,-15.9224078539418,
-21.2350540690844));
#123150=CARTESIAN_POINT('Ctrl Pts',(-16.1392442526231,-17.3849814787741,
-21.3622298757658));
#123151=CARTESIAN_POINT('Ctrl Pts',(-16.0124741552623,-20.2860474906393,
-21.4894056824473));
#123152=CARTESIAN_POINT('Ctrl Pts',(-18.3814921015747,-21.9615662752975,
-21.6165814891287));
#123153=CARTESIAN_POINT('Ctrl Pts',(-21.0759341658266,-20.8791897513666,
-21.7437572958101));
#123154=CARTESIAN_POINT('Ctrl Pts',(-21.6178065999207,-18.0222756693125,
-21.8709331024916));
#123155=CARTESIAN_POINT('Ctrl Pts',(-20.2210099178527,-16.6964452859245,
-21.9557169736125));
#123156=CARTESIAN_POINT('Ctrl Pts',(-19.3965839472885,-16.475840953354,
-21.998108909173));
#123157=CARTESIAN_POINT('Ctrl Pts',(-17.1140743056112,-17.5890877707427,
-8.67361737988404E-19));
#123158=CARTESIAN_POINT('Ctrl Pts',(-17.0606037558837,-17.6406831599911,
-2.5078829569074E-15));
#123159=CARTESIAN_POINT('Ctrl Pts',(-17.0102648206888,-17.6951284552545,
-2.007042086044E-14));
#123160=CARTESIAN_POINT('Ctrl Pts',(-16.9630512610728,-17.7520566525928,
-1.37546224410201E-14));
#123161=CARTESIAN_POINT('Ctrl Pts',(-16.9139640310005,-17.811244045856,
-7.38887994500031E-15));
#123162=CARTESIAN_POINT('Ctrl Pts',(-16.8682546395764,-17.873115719352,
2.33283173511089E-14));
#123163=CARTESIAN_POINT('Ctrl Pts',(-16.8259443403958,-17.937308752054,
1.43114686768087E-14));
#123164=CARTESIAN_POINT('Ctrl Pts',(-16.7856210013394,-17.9984871760508,
5.71806580905755E-15));
#123165=CARTESIAN_POINT('Ctrl Pts',(-16.7483849217229,-18.061774974692,
-4.47536531428885E-15));
#123166=CARTESIAN_POINT('Ctrl Pts',(-16.7142833600929,-18.1268912399334,
5.98826543907194E-15));
#123167=CARTESIAN_POINT('Ctrl Pts',(-16.6917479443229,-18.1699221757752,
1.29207969252189E-14));
#123168=CARTESIAN_POINT('Ctrl Pts',(-16.670581955631,-18.2137522504246,
3.54242763103226E-14));
#123169=CARTESIAN_POINT('Ctrl Pts',(-16.6508067523184,-18.2583061596181,
7.78543896018391E-15));
#123170=CARTESIAN_POINT('Ctrl Pts',(-16.6447946121616,-18.271851625744,
-8.45379769840918E-16));
#123171=CARTESIAN_POINT('Ctrl Pts',(-16.6389106011744,-18.2854654139231,
-1.30923055976207E-14));
#123172=CARTESIAN_POINT('Ctrl Pts',(-16.6331633226596,-18.2991259028343,
-9.75608482889356E-15));
#123173=CARTESIAN_POINT('Ctrl Pts',(-16.6020274374077,-18.3731316107767,
9.37891228514535E-15));
#123174=CARTESIAN_POINT('Ctrl Pts',(-16.5748437493431,-18.4486320984917,
1.93805730149152E-15));
#123175=CARTESIAN_POINT('Ctrl Pts',(-16.5516340690814,-18.5252437971799,
-1.49880108324396E-15));
#123176=CARTESIAN_POINT('Ctrl Pts',(-16.5281113691171,-18.6028887272984,
-4.98201100652448E-15));
#123177=CARTESIAN_POINT('Ctrl Pts',(-16.5086701130901,-18.681675875735,
-7.86786714558005E-15));
#123178=CARTESIAN_POINT('Ctrl Pts',(-16.4933735667358,-18.7612412026049,
-6.84174938925253E-15));
#123179=CARTESIAN_POINT('Ctrl Pts',(-16.4780905784648,-18.8407360068025,
-5.81654113168692E-15));
#123180=CARTESIAN_POINT('Ctrl Pts',(-16.4669445521158,-18.9210085587578,
6.00582690367431E-15));
#123181=CARTESIAN_POINT('Ctrl Pts',(-16.4600452985135,-19.0017172100912,
9.58955137519979E-15));
#123182=CARTESIAN_POINT('Ctrl Pts',(-16.4582499089088,-19.0227199854594,
1.05221423529152E-14));
#123183=CARTESIAN_POINT('Ctrl Pts',(-16.4567423723373,-19.0437523636843,
5.40618910968218E-15));
#123184=CARTESIAN_POINT('Ctrl Pts',(-16.4555251966164,-19.0648084381479,
-2.52575738102223E-15));
#123185=CARTESIAN_POINT('Ctrl Pts',(-16.4546316923203,-19.0802652803004,
-8.37958959373255E-15));
#123186=CARTESIAN_POINT('Ctrl Pts',(-16.4538946607534,-19.0957348924738,
-2.64516391872053E-16));
#123187=CARTESIAN_POINT('Ctrl Pts',(-16.4533151797917,-19.1112149436894,
-8.82627304576999E-15));
#123188=CARTESIAN_POINT('Ctrl Pts',(-16.4528674697077,-19.1231749138822,
-1.55251639105376E-14));
#123189=CARTESIAN_POINT('Ctrl Pts',(-16.4525139746189,-19.1351378160613,
-1.99942219331142E-14));
#123190=CARTESIAN_POINT('Ctrl Pts',(-16.4522551154433,-19.1470940326229,
-1.58206781009085E-14));
#123191=CARTESIAN_POINT('Ctrl Pts',(-16.450448336251,-19.23054575209,1.4416882724211E-14));
#123192=CARTESIAN_POINT('Ctrl Pts',(-16.4532433905666,-19.3137912323742,
1.21306277354053E-14));
#123193=CARTESIAN_POINT('Ctrl Pts',(-16.4606965224471,-19.3964498394684,
8.65973959207622E-15));
#123194=CARTESIAN_POINT('Ctrl Pts',(-16.4681353636814,-19.4789499568243,
5.1686934198692E-15));
#123195=CARTESIAN_POINT('Ctrl Pts',(-16.4802140623254,-19.560866453353,
1.07908903342738E-14));
#123196=CARTESIAN_POINT('Ctrl Pts',(-16.4970379007565,-19.6418365052423,
-5.4678483962789E-15));
#123197=CARTESIAN_POINT('Ctrl Pts',(-16.5134756240274,-19.7209482556099,
-2.11473992649223E-14));
#123198=CARTESIAN_POINT('Ctrl Pts',(-16.5344429618587,-19.7991574576156,
-2.06891388249104E-14));
#123199=CARTESIAN_POINT('Ctrl Pts',(-16.5596742522225,-19.8762376297952,
-9.24260668000443E-15));
#123200=CARTESIAN_POINT('Ctrl Pts',(-16.5700716763688,-19.9080011754509,
-4.62300519733931E-15));
#123201=CARTESIAN_POINT('Ctrl Pts',(-16.5811937949009,-19.9395729260017,
5.7031583328198E-15));
#123202=CARTESIAN_POINT('Ctrl Pts',(-16.593024502045,-19.9709365575929,
-9.27036225562006E-15));
#123203=CARTESIAN_POINT('Ctrl Pts',(-16.599575769931,-19.9883042051838,
-1.76032698893732E-14));
#123204=CARTESIAN_POINT('Ctrl Pts',(-16.6063465654584,-20.005613174688,
-7.16344049788605E-15));
#123205=CARTESIAN_POINT('Ctrl Pts',(-16.6133217610784,-20.0228306160632,
-1.08524300657109E-14));
#123206=CARTESIAN_POINT('Ctrl Pts',(-16.6442809363235,-20.0992496606094,
-2.70898603106819E-14));
#123207=CARTESIAN_POINT('Ctrl Pts',(-16.6792960167752,-20.1739619594251,
-1.89218150302011E-14));
#123208=CARTESIAN_POINT('Ctrl Pts',(-16.7180389842821,-20.246743899253,
-5.16253706450698E-15));
#123209=CARTESIAN_POINT('Ctrl Pts',(-16.7588459173261,-20.3234031728317,
9.3297429751869E-15));
#123210=CARTESIAN_POINT('Ctrl Pts',(-16.803788552284,-20.3979217843379,
7.49644749155628E-15));
#123211=CARTESIAN_POINT('Ctrl Pts',(-16.8525440995263,-20.4700328123178,
-7.60502771868232E-15));
#123212=CARTESIAN_POINT('Ctrl Pts',(-16.9012996467686,-20.5421438402977,
-2.27065029289209E-14));
#123213=CARTESIAN_POINT('Ctrl Pts',(-16.9538687049381,-20.6118481705157,
-1.06758067088701E-14));
#123214=CARTESIAN_POINT('Ctrl Pts',(-17.009981736112,-20.6788601850433,
4.96824803519758E-15));
#123215=CARTESIAN_POINT('Ctrl Pts',(-17.0318954596463,-20.7050302694089,
1.09555345227255E-14));
#123216=CARTESIAN_POINT('Ctrl Pts',(-17.0543502078806,-20.7307894693846,
-3.37511572030332E-15));
#123217=CARTESIAN_POINT('Ctrl Pts',(-17.0773318266369,-20.7561195433156,
-1.82909243306995E-14));
#123218=CARTESIAN_POINT('Ctrl Pts',(-17.0864635878594,-20.7661844647356,
-2.42397533361988E-14));
#123219=CARTESIAN_POINT('Ctrl Pts',(-17.0956793012105,-20.776182428681,
-2.66883060451255E-15));
#123220=CARTESIAN_POINT('Ctrl Pts',(-17.1049757714685,-20.7861097474567,
-2.1094237467878E-15));
#123221=CARTESIAN_POINT('Ctrl Pts',(-17.1654853800672,-20.8507254733048,
1.12948522341814E-15));
#123222=CARTESIAN_POINT('Ctrl Pts',(-17.2292147782235,-20.9121401114294,
-1.67082407375528E-14));
#123223=CARTESIAN_POINT('Ctrl Pts',(-17.2958558788046,-20.9700792980957,
-2.3037127760972E-15));
#123224=CARTESIAN_POINT('Ctrl Pts',(-17.3510487696017,-21.018065168297,
9.62627535178633E-15));
#123225=CARTESIAN_POINT('Ctrl Pts',(-17.4082400170084,-21.063667078019,
-2.71614749528282E-14));
#123226=CARTESIAN_POINT('Ctrl Pts',(-17.4672777570143,-21.1067151950334,
-5.6621374255883E-15));
#123227=CARTESIAN_POINT('Ctrl Pts',(-17.4867746670186,-21.1209316142798,
1.51004478036007E-15));
#123228=CARTESIAN_POINT('Ctrl Pts',(-17.5064731111025,-21.1348693857667,
-3.24941689518543E-14));
#123229=CARTESIAN_POINT('Ctrl Pts',(-17.5263680478785,-21.1485219846966,
-2.4008572907519E-14));
#123230=CARTESIAN_POINT('Ctrl Pts',(-17.5422931318004,-21.1594503322534,
-1.70799939015646E-14));
#123231=CARTESIAN_POINT('Ctrl Pts',(-17.5583454808324,-21.1701967133747,
-2.25387075678082E-14));
#123232=CARTESIAN_POINT('Ctrl Pts',(-17.574506564613,-21.1807476004758,
-2.41195952099815E-14));
#123233=CARTESIAN_POINT('Ctrl Pts',(-17.6490343637846,-21.2294036439462,
-3.11874514914714E-14));
#123234=CARTESIAN_POINT('Ctrl Pts',(-17.7259442979181,-21.2739559986071,
-3.29361491763752E-14));
#123235=CARTESIAN_POINT('Ctrl Pts',(-17.804955500985,-21.3141140597646,
-1.57651669496772E-14));
#123236=CARTESIAN_POINT('Ctrl Pts',(-17.8827967354047,-21.3536774752179,
1.60414781620485E-15));
#123237=CARTESIAN_POINT('Ctrl Pts',(-17.9626781499771,-21.3889764950412,
-4.80502357855522E-15));
#123238=CARTESIAN_POINT('Ctrl Pts',(-18.0443636118602,-21.4196958725292,
4.32986979603811E-15));
#123239=CARTESIAN_POINT('Ctrl Pts',(-18.0530583776972,-21.4229657052236,
5.14226553249037E-15));
#123240=CARTESIAN_POINT('Ctrl Pts',(-18.0617736083461,-21.4261836096314,
1.19766446651732E-14));
#123241=CARTESIAN_POINT('Ctrl Pts',(-18.0705088883292,-21.4293497159892,
-1.11022302462516E-16));
#123242=CARTESIAN_POINT('Ctrl Pts',(-19.3965839546295,-21.4281590740807,
-0.00189110722368073));
#123243=CARTESIAN_POINT('Ctrl Pts',(-20.2210099343281,-21.207554739066,
-0.0442830427841589));
#123244=CARTESIAN_POINT('Ctrl Pts',(-21.6178066866466,-19.8817246731204,
-0.129066913905115));
#123245=CARTESIAN_POINT('Ctrl Pts',(-21.0759341432978,-17.0248100445211,
-0.25624272058655));
#123246=CARTESIAN_POINT('Ctrl Pts',(-18.381492106794,-15.9424338299618,
-0.383418527267984));
#123247=CARTESIAN_POINT('Ctrl Pts',(-16.0124741472572,-17.6179524340247,
-0.510594333949419));
#123248=CARTESIAN_POINT('Ctrl Pts',(-16.1392442377966,-20.5190185688902,
-0.637770140630851));
#123249=CARTESIAN_POINT('Ctrl Pts',(-18.6470824574045,-21.9815921336573,
-0.764945947312287));
#123250=CARTESIAN_POINT('Ctrl Pts',(-21.2343815212355,-20.6651440828081,
-0.892121753993719));
#123251=CARTESIAN_POINT('Ctrl Pts',(-21.5278813636115,-17.7767637319101,
-1.01929756067515));
#123252=CARTESIAN_POINT('Ctrl Pts',(-19.2580928773362,-15.966708532015,
-1.14647336735659));
#123253=CARTESIAN_POINT('Ctrl Pts',(-16.5075209349949,-16.8954112973593,
-1.27364917403802));
#123254=CARTESIAN_POINT('Ctrl Pts',(-15.7995849828837,-19.7109385580857,
-1.40082498071946));
#123255=CARTESIAN_POINT('Ctrl Pts',(-17.7838032463622,-21.8301701846349,
-1.52800078740089));
#123256=CARTESIAN_POINT('Ctrl Pts',(-20.6397625706149,-21.308867928169,
-1.65517659408233));
#123257=CARTESIAN_POINT('Ctrl Pts',(-21.7473058680115,-18.6252811563658,
-1.78235240076376));
#123258=CARTESIAN_POINT('Ctrl Pts',(-20.0903265808676,-16.2414409677205,
-1.9095282074452));
#123259=CARTESIAN_POINT('Ctrl Pts',(-17.1890026057441,-16.3443692494651,
-2.03670401412663));
#123260=CARTESIAN_POINT('Ctrl Pts',(-15.7051174484919,-18.8396375226619,
-2.16387982080806));
#123261=CARTESIAN_POINT('Ctrl Pts',(-17.000044245167,-21.4379910700896,
-2.2910556274895));
#123262=CARTESIAN_POINT('Ctrl Pts',(-19.8857677182557,-21.7556022772552,
-2.41823143417093));
#123263=CARTESIAN_POINT('Ctrl Pts',(-21.7148158522574,-19.5010823187472,
-2.54540724085237));
#123264=CARTESIAN_POINT('Ctrl Pts',(-20.8091504232289,-16.7428134580815,
-2.6725830475338));
#123265=CARTESIAN_POINT('Ctrl Pts',(-17.9996632942386,-16.0113361084815,
-2.79975885421524));
#123266=CARTESIAN_POINT('Ctrl Pts',(-15.8638845069282,-17.9777353733943,
-2.92693466089667));
#123267=CARTESIAN_POINT('Ctrl Pts',(-16.3612585490912,-20.837961957188,
-3.0541104675781));
#123268=CARTESIAN_POINT('Ctrl Pts',(-19.035475601424,-21.9679355045566,
-3.18128627425954));
#123269=CARTESIAN_POINT('Ctrl Pts',(-21.433107502224,-20.3309754148531,
-3.30846208094097));
#123270=CARTESIAN_POINT('Ctrl Pts',(-21.354475794674,-17.4288909717763,
-3.43563788762241));
#123271=CARTESIAN_POINT('Ctrl Pts',(-18.8717201908742,-15.9241645268262,
-3.56281369430384));
#123272=CARTESIAN_POINT('Ctrl Pts',(-16.2626148596744,-17.1972892000883,
-3.68998950098528));
#123273=CARTESIAN_POINT('Ctrl Pts',(-15.920852003341,-20.0802521225103,
-3.8171653076667));
#123274=CARTESIAN_POINT('Ctrl Pts',(-18.1599778302449,-21.9281137498178,
-3.94434111434815));
#123275=CARTESIAN_POINT('Ctrl Pts',(-20.9257333700864,-21.0455757300857,
-4.07151692102957));
#123276=CARTESIAN_POINT('Ctrl Pts',(-21.6807095771773,-18.2423119199819,
-4.19869272771102));
#123277=CARTESIAN_POINT('Ctrl Pts',(-19.7322626406366,-16.0901428750757,
-4.32586853439245));
#123278=CARTESIAN_POINT('Ctrl Pts',(-16.867971690476,-16.5635501154064,
-4.45304434107388));
#123279=CARTESIAN_POINT('Ctrl Pts',(-15.7156458955264,-19.2282118809307,
-4.58022014775532));
#123280=CARTESIAN_POINT('Ctrl Pts',(-17.3324726512467,-21.639466389345,
-4.70739595443675));
#123281=CARTESIAN_POINT('Ctrl Pts',(-20.2351137608509,-21.5851372885107,
-4.83457176111819));
#123282=CARTESIAN_POINT('Ctrl Pts',(-21.7605761645016,-19.1150681563997,
-4.96174756779962));
#123283=CARTESIAN_POINT('Ctrl Pts',(-20.5093427877246,-16.4953941119431,
-5.08892337448106));
#123284=CARTESIAN_POINT('Ctrl Pts',(-17.6293425934107,-16.1295034956214,
-5.21609918116249));
#123285=CARTESIAN_POINT('Ctrl Pts',(-15.7627970068714,-18.353078238177,
-5.34327498784392));
#123286=CARTESIAN_POINT('Ctrl Pts',(-16.6221457528718,-21.1261265239282,
-5.47045079452535));
#123287=CARTESIAN_POINT('Ctrl Pts',(-19.418989694155,-21.904548665486,-5.5976266012068));
#123288=CARTESIAN_POINT('Ctrl Pts',(-21.5873981063063,-19.9741906622979,
-5.72480240788822));
#123289=CARTESIAN_POINT('Ctrl Pts',(-21.1379908577814,-17.1060361707592,
-5.85197821456966));
#123290=CARTESIAN_POINT('Ctrl Pts',(-18.4830712057421,-15.9314389191122,
-5.97915402125109));
#123291=CARTESIAN_POINT('Ctrl Pts',(-16.0583631480371,-17.5280189820156,
-6.10632982793253));
#123292=CARTESIAN_POINT('Ctrl Pts',(-16.0883858332559,-20.43101324669,-6.23350563461397));
#123293=CARTESIAN_POINT('Ctrl Pts',(-18.5455953111282,-21.9771046554413,
-6.3606814412954));
#123294=CARTESIAN_POINT('Ctrl Pts',(-21.1756543973266,-20.7478503019954,
-6.48785724797683));
#123295=CARTESIAN_POINT('Ctrl Pts',(-21.5656471201409,-17.8710147595092,
-6.61503305465826));
#123296=CARTESIAN_POINT('Ctrl Pts',(-19.3577793620672,-15.9859160816625,
-6.74220886133971));
#123297=CARTESIAN_POINT('Ctrl Pts',(-16.5776327554104,-16.8220153029603,
-6.86938466802113));
#123298=CARTESIAN_POINT('Ctrl Pts',(-15.7758192564191,-19.6122432820323,
-6.99656047470258));
#123299=CARTESIAN_POINT('Ctrl Pts',(-17.6879529842593,-21.7967390291592,
-7.123736281384));
#123300=CARTESIAN_POINT('Ctrl Pts',(-20.5597699240417,-21.3713632814495,
-7.25091208806544));
#123301=CARTESIAN_POINT('Ctrl Pts',(-21.7565562785773,-18.7263718856303,
-7.37808789474687));
#123302=CARTESIAN_POINT('Ctrl Pts',(-20.1803348485183,-16.2883802806852,
-7.50526370142831));
#123303=CARTESIAN_POINT('Ctrl Pts',(-17.2771909646086,-16.2940944453266,
-7.63243950810973));
#123304=CARTESIAN_POINT('Ctrl Pts',(-15.7105789509042,-18.7382719881573,
-7.75961531479118));
#123305=CARTESIAN_POINT('Ctrl Pts',(-16.9177680950714,-21.3785317163971,
-7.8867911214726));
#123306=CARTESIAN_POINT('Ctrl Pts',(-19.7912372839452,-21.7925992023863,
-8.01396692815404));
#123307=CARTESIAN_POINT('Ctrl Pts',(-21.6947568843456,-19.6005932276563,
-8.14114273483548));
#123308=CARTESIAN_POINT('Ctrl Pts',(-20.8819658086561,-16.8135432227874,
-8.26831854151691));
#123309=CARTESIAN_POINT('Ctrl Pts',(-18.098549421318,-15.9883945834145,
-8.39549434819835));
#123310=CARTESIAN_POINT('Ctrl Pts',(-15.8981194994098,-17.8821699716618,
-8.52267015487978));
#123311=CARTESIAN_POINT('Ctrl Pts',(-16.2994339221984,-20.7574480097691,
-8.64984596156122));
#123312=CARTESIAN_POINT('Ctrl Pts',(-18.9343116151575,-21.9763395576547,
-8.77702176824265));
#123313=CARTESIAN_POINT('Ctrl Pts',(-21.3854158339506,-20.4205872730748,
-8.90419757492408));
#123314=CARTESIAN_POINT('Ctrl Pts',(-21.4040105905201,-17.5174973162549,
-9.03137338160553));
#123315=CARTESIAN_POINT('Ctrl Pts',(-18.9730363498343,-15.9304745364933,
-9.15854918828694));
#123316=CARTESIAN_POINT('Ctrl Pts',(-16.3227610944446,-17.1155138324785,
-9.28572499496839));
#123317=CARTESIAN_POINT('Ctrl Pts',(-15.884647876537,-19.985415201978,-9.41290080164982));
#123318=CARTESIAN_POINT('Ctrl Pts',(-18.060638381169,-21.9072222646439,
-9.54007660833126));
#123319=CARTESIAN_POINT('Ctrl Pts',(-20.8543963775427,-21.1177963212788,
-9.66725241501268));
#123320=CARTESIAN_POINT('Ctrl Pts',(-21.7028223041627,-18.3413866776205,
-9.79442822169412));
#123321=CARTESIAN_POINT('Ctrl Pts',(-19.8275380326068,-16.1251768583083,
-9.92160402837556));
#123322=CARTESIAN_POINT('Ctrl Pts',(-16.949000488759,-16.5024018190668,
-10.048779835057));
#123323=CARTESIAN_POINT('Ctrl Pts',(-15.7080892069104,-19.1269810716216,
-10.1759556417385));
#123324=CARTESIAN_POINT('Ctrl Pts',(-17.2432632685167,-21.5910260515137,
-10.3031314484199));
#123325=CARTESIAN_POINT('Ctrl Pts',(-20.1460957557023,-21.6339284255716,
-10.4303072551013));
#123326=CARTESIAN_POINT('Ctrl Pts',(-21.7534180315782,-19.2163279284187,
-10.5574830617828));
#123327=CARTESIAN_POINT('Ctrl Pts',(-20.5906116696995,-16.5562229629832,
-10.6846588684642));
#123328=CARTESIAN_POINT('Ctrl Pts',(-17.7244793351877,-16.0940947303175,
-10.8118346751456));
#123329=CARTESIAN_POINT('Ctrl Pts',(-15.7845195527222,-18.2539172009796,
-10.9390104818271));
#123330=CARTESIAN_POINT('Ctrl Pts',(-16.5505250152316,-21.0541873118379,
-11.0661862885085));
#123331=CARTESIAN_POINT('Ctrl Pts',(-19.3197332545243,-21.9258310405445,
-11.1933620951899));
#123332=CARTESIAN_POINT('Ctrl Pts',(-21.5515675874969,-20.0691693663223,
-11.3205379018714));
#123333=CARTESIAN_POINT('Ctrl Pts',(-21.1984585369079,-17.1875741378502,
-11.4477137085528));
#123334=CARTESIAN_POINT('Ctrl Pts',(-18.5843617402537,-15.9247301252809,
-11.5748895152342));
#123335=CARTESIAN_POINT('Ctrl Pts',(-16.1075487593188,-17.4392183292074,
-11.7020653219157));
#123336=CARTESIAN_POINT('Ctrl Pts',(-16.04034177576,-20.3415898222665,-11.8292411285971));
#123337=CARTESIAN_POINT('Ctrl Pts',(-18.4443990256569,-21.9690989010672,
-11.9564169352785));
#123338=CARTESIAN_POINT('Ctrl Pts',(-21.1141471948498,-20.828607000416,
-12.08359274196));
#123339=CARTESIAN_POINT('Ctrl Pts',(-21.6002580413636,-17.9664446522494,
-12.2107685486414));
#123340=CARTESIAN_POINT('Ctrl Pts',(-19.4567550349637,-16.0084681651805,
-12.3379443553228));
#123341=CARTESIAN_POINT('Ctrl Pts',(-16.6501691432213,-16.7509994403685,
-12.4651201620043));
#123342=CARTESIAN_POINT('Ctrl Pts',(-15.7553687254437,-19.5128121195169,
-12.5922959686857));
#123343=CARTESIAN_POINT('Ctrl Pts',(-17.5932776273647,-21.7601144869345,
-12.7194717753671));
#123344=CARTESIAN_POINT('Ctrl Pts',(-20.4777285049632,-21.4311461038309,
-12.8466475820486));
#123345=CARTESIAN_POINT('Ctrl Pts',(-21.7624167072548,-18.8277150436234,
-12.97382338873));
#123346=CARTESIAN_POINT('Ctrl Pts',(-20.2687205453794,-16.3383077168971,
-13.1009991954114));
#123347=CARTESIAN_POINT('Ctrl Pts',(-17.3670135386182,-16.2468008358791,
-13.2281750020929));
#123348=CARTESIAN_POINT('Ctrl Pts',(-15.7194317654263,-18.6371462843459,
-13.3553508087743));
#123349=CARTESIAN_POINT('Ctrl Pts',(-16.8375292422496,-21.3163504748999,
-13.4825266154557));
#123350=CARTESIAN_POINT('Ctrl Pts',(-19.6955209310585,-21.8264098528738,
-13.6097024221372));
#123351=CARTESIAN_POINT('Ctrl Pts',(-21.6713768443407,-19.699376596832,
-13.7368782288186));
#123352=CARTESIAN_POINT('Ctrl Pts',(-20.9523718171085,-16.8866717006199,
-13.8640540355001));
#123353=CARTESIAN_POINT('Ctrl Pts',(-18.1981483353623,-15.9687773303578,
-13.9912298421815));
#123354=CARTESIAN_POINT('Ctrl Pts',(-15.9355354972161,-17.7878045998115,
-14.1184056488629));
#123355=CARTESIAN_POINT('Ctrl Pts',(-16.240340148078,-20.6749088908223,
-14.2455814555443));
#123356=CARTESIAN_POINT('Ctrl Pts',(-18.8329229390928,-21.9813512102896,
-14.3727572622258));
#123357=CARTESIAN_POINT('Ctrl Pts',(-21.3347500733399,-20.5085518170573,
-14.4999330689072));
#123358=CARTESIAN_POINT('Ctrl Pts',(-21.450550436052,-17.6077127421763,
-14.6271088755887));
#123359=CARTESIAN_POINT('Ctrl Pts',(-19.0740843818219,-15.9401737904716,
-14.7542846822701));
#123360=CARTESIAN_POINT('Ctrl Pts',(-16.3856120152874,-17.0357984509923,
-14.8814604889515));
#123361=CARTESIAN_POINT('Ctrl Pts',(-15.85163986733,-19.8894190998463,-15.008636295633));
#123362=CARTESIAN_POINT('Ctrl Pts',(-17.9620542416513,-21.8830159073825,
-15.1358121023144));
#123363=CARTESIAN_POINT('Ctrl Pts',(-20.7806809369002,-21.1875875392591,
-15.2629879089958));
#123364=CARTESIAN_POINT('Ctrl Pts',(-21.7216049038886,-18.4411463600769,
-15.3901637156773));
#123365=CARTESIAN_POINT('Ctrl Pts',(-19.9215868032322,-16.1633816883713,
-15.5173395223587));
#123366=CARTESIAN_POINT('Ctrl Pts',(-17.0320315205603,-16.4440012364127,
-15.6445153290401));
#123367=CARTESIAN_POINT('Ctrl Pts',(-15.7039266816969,-19.0255539860864,
-15.7716911357216));
#123368=CARTESIAN_POINT('Ctrl Pts',(-17.1557260448163,-21.5396255188012,
-15.898866942403));
#123369=CARTESIAN_POINT('Ctrl Pts',(-20.0554938030874,-21.6797112441684,
-16.0260427490844));
#123370=CARTESIAN_POINT('Ctrl Pts',(-21.7428730181815,-19.3172912038646,
-16.1532185557659));
#123371=CARTESIAN_POINT('Ctrl Pts',(-20.6697979908152,-16.6197391565441,
-16.2803943624473));
#123372=CARTESIAN_POINT('Ctrl Pts',(-17.8207484560495,-16.0618916766609,
-16.4075701691287));
#123373=CARTESIAN_POINT('Ctrl Pts',(-15.8095505300749,-18.1555392030885,
-16.5347459758102));
#123374=CARTESIAN_POINT('Ctrl Pts',(-16.4813534809519,-20.9798900767501,
-16.6619217824916));
#123375=CARTESIAN_POINT('Ctrl Pts',(-19.2198197980441,-21.9437776700467,
-16.789097589173));
#123376=CARTESIAN_POINT('Ctrl Pts',(-21.5125766038083,-20.1628949417396,
-16.9162733958545));
#123377=CARTESIAN_POINT('Ctrl Pts',(-21.2561618334919,-17.2710912610025,
-17.0434492025359));
#123378=CARTESIAN_POINT('Ctrl Pts',(-18.6858201239648,-15.9214170193332,
-17.1706250092173));
#123379=CARTESIAN_POINT('Ctrl Pts',(-16.1596804603196,-17.3521145632324,
-17.2978008158988));
#123380=CARTESIAN_POINT('Ctrl Pts',(-15.9953191940406,-20.2506076952764,
-17.4249766225802));
#123381=CARTESIAN_POINT('Ctrl Pts',(-18.3435275855282,-21.9577088675884,
-17.5521524292616));
#123382=CARTESIAN_POINT('Ctrl Pts',(-21.0499701818423,-20.9072587092191,
-17.6793282359431));
#123383=CARTESIAN_POINT('Ctrl Pts',(-21.631653881637,-18.0629800421848,
-17.8065040426245));
#123384=CARTESIAN_POINT('Ctrl Pts',(-19.5549199937129,-16.0343220076414,
-17.933679849306));
#123385=CARTESIAN_POINT('Ctrl Pts',(-16.725042963598,-16.6824524395731,
-18.0608556559873));
#123386=CARTESIAN_POINT('Ctrl Pts',(-15.7382593244464,-19.4127518941776,
-18.1880314626688));
#123387=CARTESIAN_POINT('Ctrl Pts',(-17.4998818184781,-21.7203400833824,
-18.3152072693502));
#123388=CARTESIAN_POINT('Ctrl Pts',(-20.3937311460449,-21.4881480686078,
-18.4423830760317));
#123389=CARTESIAN_POINT('Ctrl Pts',(-21.7648801616449,-18.9291976120636,
-18.5695588827131));
#123390=CARTESIAN_POINT('Ctrl Pts',(-20.3553847465806,-16.3911669310282,
-18.6967346893946));
#123391=CARTESIAN_POINT('Ctrl Pts',(-17.4583694610031,-16.2025416478318,
-18.823910496076));
#123392=CARTESIAN_POINT('Ctrl Pts',(-15.7316660204183,-18.5363737515732,
-18.9510863027574));
#123393=CARTESIAN_POINT('Ctrl Pts',(-16.7594176601915,-21.2515171426226,
-19.0782621094388));
#123394=CARTESIAN_POINT('Ctrl Pts',(-19.5987260404249,-21.8569962774213,
-19.2054379161203));
#123395=CARTESIAN_POINT('Ctrl Pts',(-21.6447019493503,-19.7973216359904,
-19.3326137228017));
#123396=CARTESIAN_POINT('Ctrl Pts',(-21.0202894786101,-16.9621168526002,
-19.4597895294832));
#123397=CARTESIAN_POINT('Ctrl Pts',(-18.2983483137461,-15.9525063653534,
-19.5869653361646));
#123398=CARTESIAN_POINT('Ctrl Pts',(-15.9760905326363,-17.6947450904228,
-19.714141142846));
#123399=CARTESIAN_POINT('Ctrl Pts',(-16.184043510336,-20.5904372147467,
-19.8413169495275));
#123400=CARTESIAN_POINT('Ctrl Pts',(-18.7314233036429,-21.9829647838468,
-19.9684927562089));
#123401=CARTESIAN_POINT('Ctrl Pts',(-21.2811670472796,-20.5947704862203,
-20.0956685628903));
#123402=CARTESIAN_POINT('Ctrl Pts',(-21.49404313672,-17.6994358448221,-20.2228443695718));
#123403=CARTESIAN_POINT('Ctrl Pts',(-19.1747509237061,-15.9532518137242,
-20.3500201762532));
#123404=CARTESIAN_POINT('Ctrl Pts',(-16.4510971561478,-16.9582316928714,
-20.4771959829346));
#123405=CARTESIAN_POINT('Ctrl Pts',(-15.8218649356901,-19.7923729967134,
-20.6043717896161));
#123406=CARTESIAN_POINT('Ctrl Pts',(-17.8643361189216,-21.8555189367891,
-20.7315475962975));
#123407=CARTESIAN_POINT('Ctrl Pts',(-20.704669493102,-21.2548766742021,
-20.8587234029789));
#123408=CARTESIAN_POINT('Ctrl Pts',(-21.7370367735022,-18.5414683255483,
-20.9858992096604));
#123409=CARTESIAN_POINT('Ctrl Pts',(-20.0143025609789,-16.2047352065647,
-21.1130750163418));
#123410=CARTESIAN_POINT('Ctrl Pts',(-17.1169733783673,-16.3883740006192,
-21.2402508230232));
#123411=CARTESIAN_POINT('Ctrl Pts',(-15.7031596587772,-18.9241212228848,
-21.3674266297047));
#123412=CARTESIAN_POINT('Ctrl Pts',(-17.0699655881192,-21.4851744179203,
-21.4946024363861));
#123413=CARTESIAN_POINT('Ctrl Pts',(-19.963397156019,-21.7227196345909,
-21.6217782430676));
#123414=CARTESIAN_POINT('Ctrl Pts',(-21.7289768951727,-19.4172948235399,
-21.748954049749));
#123415=CARTESIAN_POINT('Ctrl Pts',(-20.7467658607354,-16.6869340105708,
-21.8761298564304));
#123416=CARTESIAN_POINT('Ctrl Pts',(-17.9181415113151,-16.0308544058051,
-22.0033056631118));
#123417=CARTESIAN_POINT('Ctrl Pts',(-15.8372814923396,-18.0626244799711,
-22.1305001261329));
#123418=CARTESIAN_POINT('Ctrl Pts',(-16.2233207480177,-19.9500078885456,
-22.2153026535935));
#123419=CARTESIAN_POINT('Ctrl Pts',(-16.7733104792501,-20.6030838137515,
-22.2577132454937));
#123420=CARTESIAN_POINT('Ctrl Pts',(-19.3578031896578,-21.2832305070458,
0.0847272843464291));
#123421=CARTESIAN_POINT('Ctrl Pts',(-20.1339758575579,-21.0755380525683,
0.042335348785951));
#123422=CARTESIAN_POINT('Ctrl Pts',(-21.4490186733577,-19.8273082723234,
-0.0424485223350051));
#123423=CARTESIAN_POINT('Ctrl Pts',(-20.9388617059771,-17.1376076759719,
-0.169624329016439));
#123424=CARTESIAN_POINT('Ctrl Pts',(-18.4021242480669,-16.1185824938284,
-0.296800135697873));
#123425=CARTESIAN_POINT('Ctrl Pts',(-16.1717639304198,-17.6960336866052,
-0.423975942379309));
#123426=CARTESIAN_POINT('Ctrl Pts',(-16.2911142199628,-20.4273016198123,
-0.551151749060742));
#123427=CARTESIAN_POINT('Ctrl Pts',(-18.6521697052435,-21.8042713584183,
-0.678327555742178));
#123428=CARTESIAN_POINT('Ctrl Pts',(-21.0880352243816,-20.5648744678046,
-0.80550336242361));
#123429=CARTESIAN_POINT('Ctrl Pts',(-21.3643566423075,-17.8455498248734,
-0.932679169105046));
#123430=CARTESIAN_POINT('Ctrl Pts',(-19.2274179378702,-16.1414364076047,
-1.05985497578648));
#123431=CARTESIAN_POINT('Ctrl Pts',(-16.6378358343089,-17.0157825839918,
-1.18703078246792));
#123432=CARTESIAN_POINT('Ctrl Pts',(-15.9713350808349,-19.6665181980038,
-1.31420658914935));
#123433=CARTESIAN_POINT('Ctrl Pts',(-17.8394178695693,-21.6617120734788,
-1.44138239583079));
#123434=CARTESIAN_POINT('Ctrl Pts',(-20.5282190751429,-21.1709214225929,
-1.56855820251222));
#123435=CARTESIAN_POINT('Ctrl Pts',(-21.5709383211685,-18.6444038752278,
-1.69573400919365));
#123436=CARTESIAN_POINT('Ctrl Pts',(-20.0109413467548,-16.4000888674147,
-1.82290981587509));
#123437=CARTESIAN_POINT('Ctrl Pts',(-17.2794306645736,-16.4969927993764,
-1.95008562255652));
#123438=CARTESIAN_POINT('Ctrl Pts',(-15.882396692181,-18.8462140520133,
-2.07726142923796));
#123439=CARTESIAN_POINT('Ctrl Pts',(-17.1015319587312,-21.2924870403926,
-2.20443723591939));
#123440=CARTESIAN_POINT('Ctrl Pts',(-19.8183552298129,-21.5915085948938,
-2.33161304260083));
#123441=CARTESIAN_POINT('Ctrl Pts',(-21.5403499326061,-19.4689447576054,
-2.45878884928226));
#123442=CARTESIAN_POINT('Ctrl Pts',(-20.6876927267632,-16.8721162331674,
-2.5859646559637));
#123443=CARTESIAN_POINT('Ctrl Pts',(-18.0426437180737,-16.1834519504684,
-2.71314046264513));
#123444=CARTESIAN_POINT('Ctrl Pts',(-16.0318711803166,-18.0347586792573,
-2.84031626932657));
#123445=CARTESIAN_POINT('Ctrl Pts',(-16.5001341253916,-20.7275773834348,
-2.967492076008));
#123446=CARTESIAN_POINT('Ctrl Pts',(-19.0178303590937,-21.7914140461736,
-3.09466788268943));
#123447=CARTESIAN_POINT('Ctrl Pts',(-21.2751298558503,-20.2502645538495,
-3.22184368937087));
#123448=CARTESIAN_POINT('Ctrl Pts',(-21.201100429639,-17.5180379135899,
-3.3490194960523));
#123449=CARTESIAN_POINT('Ctrl Pts',(-18.8636594850319,-16.1013824854533,
-3.47619530273374));
#123450=CARTESIAN_POINT('Ctrl Pts',(-16.40726401034,-17.2999916978614,-3.60337110941517));
#123451=CARTESIAN_POINT('Ctrl Pts',(-16.0855043927131,-20.0142159921659,
-3.73054691609661));
#123452=CARTESIAN_POINT('Ctrl Pts',(-18.1935751105569,-21.7539230422786,
-3.85772272277804));
#123453=CARTESIAN_POINT('Ctrl Pts',(-20.7974521219332,-20.9230396080263,
-3.98489852945948));
#123454=CARTESIAN_POINT('Ctrl Pts',(-21.5082398837079,-18.2838496699412,
-4.11207433614091));
#123455=CARTESIAN_POINT('Ctrl Pts',(-19.6738347409324,-16.2576461895902,
-4.23925014282234));
#123456=CARTESIAN_POINT('Ctrl Pts',(-16.9771895560713,-16.703345099837,
-4.36642594950377));
#123457=CARTESIAN_POINT('Ctrl Pts',(-15.8923089135627,-19.2120453137177,
-4.49360175618521));
#123458=CARTESIAN_POINT('Ctrl Pts',(-17.4145034676192,-21.482170092496,
-4.62077756286664));
#123459=CARTESIAN_POINT('Ctrl Pts',(-20.1472541929444,-21.4310208514753,
-4.74795336954808));
#123460=CARTESIAN_POINT('Ctrl Pts',(-21.5834319126906,-19.1055238446132,
-4.87512917622951));
#123461=CARTESIAN_POINT('Ctrl Pts',(-20.4054327082334,-16.6391782390827,
-5.00230498291095));
#123462=CARTESIAN_POINT('Ctrl Pts',(-17.6939977347856,-16.2947030492859,
-5.12948078959238));
#123463=CARTESIAN_POINT('Ctrl Pts',(-15.9367002898516,-18.3881328813199,
-5.25665659627382));
#123464=CARTESIAN_POINT('Ctrl Pts',(-16.7457517089779,-20.9988757972025,
-5.38383240295525));
#123465=CARTESIAN_POINT('Ctrl Pts',(-19.3788975305108,-21.7317372125915,
-5.51100820963669));
#123466=CARTESIAN_POINT('Ctrl Pts',(-21.4203898946547,-19.914362265377,
-5.63818401631812));
#123467=CARTESIAN_POINT('Ctrl Pts',(-20.9972862666143,-17.2140796706178,
-5.76535982299955));
#123468=CARTESIAN_POINT('Ctrl Pts',(-18.4977579643435,-16.1082311105657,
-5.89253562968099));
#123469=CARTESIAN_POINT('Ctrl Pts',(-16.2149670669532,-17.6113640023665,
-6.01971143636243));
#123470=CARTESIAN_POINT('Ctrl Pts',(-16.2432325368166,-20.3444472127417,
-6.14688724304385));
#123471=CARTESIAN_POINT('Ctrl Pts',(-18.5566225596869,-21.8000465304473,
-6.2740630497253));
#123472=CARTESIAN_POINT('Ctrl Pts',(-21.0327453747589,-20.6427399261711,
-6.40123885640672));
#123473=CARTESIAN_POINT('Ctrl Pts',(-21.3999119847184,-17.9342843787876,
-6.52841466308816));
#123474=CARTESIAN_POINT('Ctrl Pts',(-19.3212698138575,-16.1595197473112,
-6.6555904697696));
#123475=CARTESIAN_POINT('Ctrl Pts',(-16.7038440388577,-16.9466824268052,
-6.78276627645102));
#123476=CARTESIAN_POINT('Ctrl Pts',(-15.9489603525162,-19.57359951566,-6.90994208313247));
#123477=CARTESIAN_POINT('Ctrl Pts',(-17.7491776836857,-21.6302376297137,
-7.03711788981389));
#123478=CARTESIAN_POINT('Ctrl Pts',(-20.452908365107,-21.2297589486797,
-7.16429369649533));
#123479=CARTESIAN_POINT('Ctrl Pts',(-21.5796473090278,-18.7395778058964,
-7.29146950317678));
#123480=CARTESIAN_POINT('Ctrl Pts',(-20.0956814677067,-16.4442808417949,
-7.41864530985819));
#123481=CARTESIAN_POINT('Ctrl Pts',(-17.3624573952481,-16.4496605587419,
-7.54582111653964));
#123482=CARTESIAN_POINT('Ctrl Pts',(-15.8875385351148,-18.7507814003416,
-7.67299692322106));
#123483=CARTESIAN_POINT('Ctrl Pts',(-17.0240713976901,-21.236507818093,
-7.80017272990251));
#123484=CARTESIAN_POINT('Ctrl Pts',(-19.7293576227465,-21.6263401052905,
-7.92734853658393));
#123485=CARTESIAN_POINT('Ctrl Pts',(-21.5214650077943,-19.5626313341509,
-8.05452434326538));
#123486=CARTESIAN_POINT('Ctrl Pts',(-20.756246257781,-16.9387062139828,
-8.1817001499468));
#123487=CARTESIAN_POINT('Ctrl Pts',(-18.1357420810118,-16.1618531833802,
-8.30887595662825));
#123488=CARTESIAN_POINT('Ctrl Pts',(-16.06410241284,-17.9447866809843,-8.43605176330966));
#123489=CARTESIAN_POINT('Ctrl Pts',(-16.4419280683544,-20.6517758840762,
-8.56322756999113));
#123490=CARTESIAN_POINT('Ctrl Pts',(-18.9225874591253,-21.7993262135178,
-8.69040337667253));
#123491=CARTESIAN_POINT('Ctrl Pts',(-21.2302295612066,-20.3346314670524,
-8.81757918335398));
#123492=CARTESIAN_POINT('Ctrl Pts',(-21.2477359743606,-17.6014581653534,
-8.9447549900354));
#123493=CARTESIAN_POINT('Ctrl Pts',(-18.9590456510891,-16.1073231728629,
-9.07193079671685));
#123494=CARTESIAN_POINT('Ctrl Pts',(-16.4638899108517,-17.2230026087143,
-9.19910660339828));
#123495=CARTESIAN_POINT('Ctrl Pts',(-16.0514192784853,-19.9249298373897,
-9.3262824100797));
#123496=CARTESIAN_POINT('Ctrl Pts',(-18.1000499583713,-21.7342543270959,
-9.45345821676116));
#123497=CARTESIAN_POINT('Ctrl Pts',(-20.7302904540745,-20.9910331578707,
-9.58063402344258));
#123498=CARTESIAN_POINT('Ctrl Pts',(-21.5290583619236,-18.3771256229697,
-9.70780983012403));
#123499=CARTESIAN_POINT('Ctrl Pts',(-19.7635337035947,-16.2906296482662,
-9.83498563680543));
#123500=CARTESIAN_POINT('Ctrl Pts',(-17.0534757722859,-16.6457757880052,
-9.9621614434869));
#123501=CARTESIAN_POINT('Ctrl Pts',(-15.8851945148077,-19.1167395018316,
-10.0893372501683));
#123502=CARTESIAN_POINT('Ctrl Pts',(-17.3305154731838,-21.4365649476141,
-10.2165130568498));
#123503=CARTESIAN_POINT('Ctrl Pts',(-20.0634463748397,-21.4769562634529,
-10.3436888635312));
#123504=CARTESIAN_POINT('Ctrl Pts',(-21.5766927423282,-19.2008569240337,
-10.4708646702126));
#123505=CARTESIAN_POINT('Ctrl Pts',(-20.4819449561405,-16.6964468026162,
-10.598040476894));
#123506=CARTESIAN_POINT('Ctrl Pts',(-17.7835661623932,-16.2613667443784,
-10.7252162835755));
#123507=CARTESIAN_POINT('Ctrl Pts',(-15.9571514240733,-18.2947756986395,
-10.8523920902569));
#123508=CARTESIAN_POINT('Ctrl Pts',(-16.678322903506,-20.9311471574582,
-10.9795678969384));
#123509=CARTESIAN_POINT('Ctrl Pts',(-19.2854505292619,-21.7517739390354,
-11.1067437036198));
#123510=CARTESIAN_POINT('Ctrl Pts',(-21.3866565212999,-20.0037819051163,
-11.2339195103012));
#123511=CARTESIAN_POINT('Ctrl Pts',(-21.0542147974772,-17.2908452542003,
-11.3610953169827));
#123512=CARTESIAN_POINT('Ctrl Pts',(-18.5931200057406,-16.1019149796642,
-11.4882711236641));
#123513=CARTESIAN_POINT('Ctrl Pts',(-16.2612738647384,-17.5277608150597,
-11.6154469303455));
#123514=CARTESIAN_POINT('Ctrl Pts',(-16.198000478146,-20.2602577043845,
-11.742622737027));
#123515=CARTESIAN_POINT('Ctrl Pts',(-18.4613492509727,-21.7925093495675,
-11.8697985437084));
#123516=CARTESIAN_POINT('Ctrl Pts',(-20.9748381634178,-20.7187699684155,
-11.9969743503898));
#123517=CARTESIAN_POINT('Ctrl Pts',(-21.4324971430291,-18.0241287993538,
-12.1241501570713));
#123518=CARTESIAN_POINT('Ctrl Pts',(-19.4144524815328,-16.1807518667032,
-12.2513259637527));
#123519=CARTESIAN_POINT('Ctrl Pts',(-16.7721349018743,-16.879823093295,
-12.3785017704341));
#123520=CARTESIAN_POINT('Ctrl Pts',(-15.9297067826652,-19.4799880179848,
-12.5056775771156));
#123521=CARTESIAN_POINT('Ctrl Pts',(-17.6600436362941,-21.5957567068059,
-12.632853383797));
#123522=CARTESIAN_POINT('Ctrl Pts',(-20.3756687963737,-21.2860427071796,
-12.7600291904784));
#123523=CARTESIAN_POINT('Ctrl Pts',(-21.5851647292373,-18.8349893907445,
-12.8872049971599));
#123524=CARTESIAN_POINT('Ctrl Pts',(-20.1788939862666,-16.4912860458039,
-13.0143808038413));
#123525=CARTESIAN_POINT('Ctrl Pts',(-17.4470226911311,-16.4051350247055,
-13.1415566105228));
#123526=CARTESIAN_POINT('Ctrl Pts',(-15.8958731980624,-18.6555745421719,
-13.2687324172041));
#123527=CARTESIAN_POINT('Ctrl Pts',(-16.9485288917557,-21.1779660189567,
-13.3959082238856));
#123528=CARTESIAN_POINT('Ctrl Pts',(-19.6392435084281,-21.6581718323812,
-13.523084030567));
#123529=CARTESIAN_POINT('Ctrl Pts',(-21.4994533918664,-19.6556329535628,
-13.6502598372485));
#123530=CARTESIAN_POINT('Ctrl Pts',(-20.8225314316626,-17.0075545122368,
-13.7774356439299));
#123531=CARTESIAN_POINT('Ctrl Pts',(-18.2295115117883,-16.1433841200358,
-13.9046114506113));
#123532=CARTESIAN_POINT('Ctrl Pts',(-16.0993284677614,-17.8559444753405,
-14.0317872572928));
#123533=CARTESIAN_POINT('Ctrl Pts',(-16.3862930284057,-20.5740677456421,
-14.1589630639742));
#123534=CARTESIAN_POINT('Ctrl Pts',(-18.8271330203595,-21.8040445361958,
-14.2861388706557));
#123535=CARTESIAN_POINT('Ctrl Pts',(-21.1825292466206,-20.4174474826375,
-14.4133146773371));
#123536=CARTESIAN_POINT('Ctrl Pts',(-21.2915518619716,-17.686393319688,
-14.5404904840185));
#123537=CARTESIAN_POINT('Ctrl Pts',(-19.0541793835346,-16.1164547335152,
-14.6676662907));
#123538=CARTESIAN_POINT('Ctrl Pts',(-16.5230621932784,-17.1479529355545,
-14.7948420973814));
#123539=CARTESIAN_POINT('Ctrl Pts',(-16.0203432144126,-19.8345523474337,
-14.9220179040628));
#123540=CARTESIAN_POINT('Ctrl Pts',(-18.0072359077879,-21.7114647579188,
-15.0491937107442));
#123541=CARTESIAN_POINT('Ctrl Pts',(-20.6608895477009,-21.0567395247122,
-15.1763695174257));
#123542=CARTESIAN_POINT('Ctrl Pts',(-21.5467416238517,-18.4710464124499,
-15.3035453241071));
#123543=CARTESIAN_POINT('Ctrl Pts',(-19.8520778385523,-16.3265983654185,
-15.4307211307886));
#123544=CARTESIAN_POINT('Ctrl Pts',(-17.1316470321183,-16.5907933673128,
-15.55789693747));
#123545=CARTESIAN_POINT('Ctrl Pts',(-15.8812756204742,-19.0212489016859,
-15.6850727441514));
#123546=CARTESIAN_POINT('Ctrl Pts',(-17.2481017670014,-21.3881728668337,
-15.8122485508329));
#123547=CARTESIAN_POINT('Ctrl Pts',(-19.9781473170593,-21.5200594326025,
-15.9394243575143));
#123548=CARTESIAN_POINT('Ctrl Pts',(-21.5667649242067,-19.295910860703,
-16.0666001641957));
#123549=CARTESIAN_POINT('Ctrl Pts',(-20.5564965346144,-16.7562454196237,
-16.1937759708772));
#123550=CARTESIAN_POINT('Ctrl Pts',(-17.8742006914056,-16.2310485221405,
-16.3209517775586));
#123551=CARTESIAN_POINT('Ctrl Pts',(-15.9807173486685,-18.2021557242983,
-16.44812758424));
#123552=CARTESIAN_POINT('Ctrl Pts',(-16.6131999505341,-20.8611985088279,
-16.5753033909215));
#123553=CARTESIAN_POINT('Ctrl Pts',(-19.1913849660881,-21.7686701597314,
-16.7024791976029));
#123554=CARTESIAN_POINT('Ctrl Pts',(-21.349947663769,-20.0920217613478,
-16.8296550042843));
#123555=CARTESIAN_POINT('Ctrl Pts',(-21.1085407439649,-17.369474154658,
-16.9568308109658));
#123556=CARTESIAN_POINT('Ctrl Pts',(-18.688640072193,-16.0987957884381,
-17.0840066176472));
#123557=CARTESIAN_POINT('Ctrl Pts',(-16.3103543188293,-17.4457551965009,
-17.2111824243287));
#123558=CARTESIAN_POINT('Ctrl Pts',(-16.1556130495236,-20.174600723678,
-17.3383582310101));
#123559=CARTESIAN_POINT('Ctrl Pts',(-18.3663817745373,-21.7817859700398,
-17.4655340376915));
#123560=CARTESIAN_POINT('Ctrl Pts',(-20.9144174044528,-20.7928182252147,
-17.5927098443729));
#123561=CARTESIAN_POINT('Ctrl Pts',(-21.4620553977494,-18.1150140128212,
-17.7198856510544));
#123562=CARTESIAN_POINT('Ctrl Pts',(-19.506871885825,-16.2050924944522,
-17.8470614577358));
#123563=CARTESIAN_POINT('Ctrl Pts',(-16.8426263884951,-16.8152881201209,
-17.9742372644172));
#123564=CARTESIAN_POINT('Ctrl Pts',(-15.9135987878357,-19.3857842762726,
-18.1014130710987));
#123565=CARTESIAN_POINT('Ctrl Pts',(-17.5721142454945,-21.5583102826521,
-18.2285888777801));
#123566=CARTESIAN_POINT('Ctrl Pts',(-20.2965877681507,-21.339708370521,
-18.3557646844615));
#123567=CARTESIAN_POINT('Ctrl Pts',(-21.5874839986603,-18.9305322264037,
-18.482940491143));
#123568=CARTESIAN_POINT('Ctrl Pts',(-20.2604857675958,-16.5410514319824,
-18.6101162978244));
#123569=CARTESIAN_POINT('Ctrl Pts',(-17.5330315891426,-16.3634663086393,
-18.7372921045058));
#123570=CARTESIAN_POINT('Ctrl Pts',(-15.907391387167,-18.560700184086,-18.8644679111873));
#123571=CARTESIAN_POINT('Ctrl Pts',(-16.8749891483064,-21.1169273548174,
-18.9916437178687));
#123572=CARTESIAN_POINT('Ctrl Pts',(-19.5481139827311,-21.6869680461436,
-19.1188195245502));
#123573=CARTESIAN_POINT('Ctrl Pts',(-21.4743397674531,-19.7478453100669,
-19.2459953312316));
#123574=CARTESIAN_POINT('Ctrl Pts',(-20.8864739005117,-17.0785838906586,
-19.373171137913));
#123575=CARTESIAN_POINT('Ctrl Pts',(-18.323846826857,-16.1280654878871,
-19.5003469445945));
#123576=CARTESIAN_POINT('Ctrl Pts',(-16.1375098337227,-17.7683317005682,
-19.6275227512759));
#123577=CARTESIAN_POINT('Ctrl Pts',(-16.3332914095993,-20.4945401618491,
-19.7546985579573));
#123578=CARTESIAN_POINT('Ctrl Pts',(-18.7315741166155,-21.8055636679596,
-19.8818743646388));
#123579=CARTESIAN_POINT('Ctrl Pts',(-21.1320824129259,-20.4986198087347,
-20.0090501713202));
#123580=CARTESIAN_POINT('Ctrl Pts',(-21.3324989528482,-17.7727479070516,
-20.1362259780016));
#123581=CARTESIAN_POINT('Ctrl Pts',(-19.1489539543349,-16.1287673054729,
-20.2634017846831));
#123582=CARTESIAN_POINT('Ctrl Pts',(-16.5847145159137,-17.0749261277227,
-20.3905775913645));
#123583=CARTESIAN_POINT('Ctrl Pts',(-15.9923109972134,-19.7431863126012,
-20.5177533980459));
#123584=CARTESIAN_POINT('Ctrl Pts',(-17.9152371863878,-21.6855771736479,
-20.6449292047274));
#123585=CARTESIAN_POINT('Ctrl Pts',(-20.5893270222873,-21.1200902544022,
-20.7721050114088));
#123586=CARTESIAN_POINT('Ctrl Pts',(-21.5612702725159,-18.5654965747524,
-20.8992808180902));
#123587=CARTESIAN_POINT('Ctrl Pts',(-19.9393669813241,-16.3655314792863,
-21.0264566247717));
#123588=CARTESIAN_POINT('Ctrl Pts',(-17.2116172781004,-16.5384219706357,
-21.1536324314531));
#123589=CARTESIAN_POINT('Ctrl Pts',(-15.8805534910891,-18.9257529561851,
-21.2808082381345));
#123590=CARTESIAN_POINT('Ctrl Pts',(-17.1673608343839,-21.3369087663789,
-21.407984044816));
#123591=CARTESIAN_POINT('Ctrl Pts',(-19.8914410486737,-21.560550559712,
-21.5351598514974));
#123592=CARTESIAN_POINT('Ctrl Pts',(-21.5536821355334,-19.3900613098573,
-21.6623356581788));
#123593=CARTESIAN_POINT('Ctrl Pts',(-20.6289595069245,-16.8195073866206,
-21.7895114648603));
#123594=CARTESIAN_POINT('Ctrl Pts',(-17.965893371406,-16.2018278499181,
-21.9166872715417));
#123595=CARTESIAN_POINT('Ctrl Pts',(-16.006825229175,-18.1146792615168,
-22.0438817345628));
#123596=CARTESIAN_POINT('Ctrl Pts',(-16.3702697667955,-19.8915948993761,
-22.1286842620234));
#123597=CARTESIAN_POINT('Ctrl Pts',(-16.8880688264085,-20.506446560642,
-22.1710948539236));
#123598=CARTESIAN_POINT('Ctrl Pts',(-19.3190224246859,-21.138301940011,
0.171345675916539));
#123599=CARTESIAN_POINT('Ctrl Pts',(-20.0469417807877,-20.9435213660705,
0.128953740356061));
#123600=CARTESIAN_POINT('Ctrl Pts',(-21.2802306600689,-19.7728918715264,
0.0441698692351047));
#123601=CARTESIAN_POINT('Ctrl Pts',(-20.8017892686562,-17.2504053074226,
-0.0830059374463295));
#123602=CARTESIAN_POINT('Ctrl Pts',(-18.42275638934,-16.2947311576948,-0.210181744127763));
#123603=CARTESIAN_POINT('Ctrl Pts',(-16.3310537135823,-17.7741149391859,
-0.337357550809198));
#123604=CARTESIAN_POINT('Ctrl Pts',(-16.4429842021291,-20.3355846707344,
-0.464533357490632));
#123605=CARTESIAN_POINT('Ctrl Pts',(-18.6572569530825,-21.6269505831793,
-0.591709164172067));
#123606=CARTESIAN_POINT('Ctrl Pts',(-20.9416889275276,-20.4646048528009,
-0.718884970853501));
#123607=CARTESIAN_POINT('Ctrl Pts',(-21.2008319210033,-17.9143359178367,
-0.846060777534935));
#123608=CARTESIAN_POINT('Ctrl Pts',(-19.1967429984043,-16.3161642831945,
-0.973236584216371));
#123609=CARTESIAN_POINT('Ctrl Pts',(-16.7681507336229,-17.1361538706243,
-1.1004123908978));
#123610=CARTESIAN_POINT('Ctrl Pts',(-16.1430851787862,-19.6220978379218,
-1.22758819757924));
#123611=CARTESIAN_POINT('Ctrl Pts',(-17.8950324927765,-21.4932539623228,
-1.35476400426067));
#123612=CARTESIAN_POINT('Ctrl Pts',(-20.4166755796707,-21.0329749170169,
-1.48193981094211));
#123613=CARTESIAN_POINT('Ctrl Pts',(-21.3945707743255,-18.6635265940897,
-1.60911561762354));
#123614=CARTESIAN_POINT('Ctrl Pts',(-19.9315561126419,-16.558736767109,
-1.73629142430498));
#123615=CARTESIAN_POINT('Ctrl Pts',(-17.369858723403,-16.6496163492876,
-1.86346723098641));
#123616=CARTESIAN_POINT('Ctrl Pts',(-16.0596759358701,-18.8527905813645,
-1.99064303766784));
#123617=CARTESIAN_POINT('Ctrl Pts',(-17.2030196722955,-21.1469830106956,
-2.11781884434928));
#123618=CARTESIAN_POINT('Ctrl Pts',(-19.7509427413702,-21.4274149125326,
-2.24499465103071));
#123619=CARTESIAN_POINT('Ctrl Pts',(-21.3658840129548,-19.4368071964635,
-2.37217045771215));
#123620=CARTESIAN_POINT('Ctrl Pts',(-20.5662350302976,-17.0014190082534,
-2.49934626439358));
#123621=CARTESIAN_POINT('Ctrl Pts',(-18.0856241419088,-16.3555677924553,
-2.62652207107501));
#123622=CARTESIAN_POINT('Ctrl Pts',(-16.1998578537051,-18.0917819851203,
-2.75369787775646));
#123623=CARTESIAN_POINT('Ctrl Pts',(-16.639009701692,-20.6171928096815,
-2.88087368443788));
#123624=CARTESIAN_POINT('Ctrl Pts',(-19.0001851167635,-21.6148925877907,
-3.00804949111932));
#123625=CARTESIAN_POINT('Ctrl Pts',(-21.1171522094764,-20.169553692846,
-3.13522529780075));
#123626=CARTESIAN_POINT('Ctrl Pts',(-21.0477250646041,-17.6071848554035,
-3.26240110448218));
#123627=CARTESIAN_POINT('Ctrl Pts',(-18.8555987791894,-16.2786004440803,
-3.38957691116362));
#123628=CARTESIAN_POINT('Ctrl Pts',(-16.5519131610055,-17.4026941956347,
-3.51675271784505));
#123629=CARTESIAN_POINT('Ctrl Pts',(-16.2501567820852,-19.9481798618215,
-3.64392852452649));
#123630=CARTESIAN_POINT('Ctrl Pts',(-18.2271723908689,-21.5797323347394,
-3.77110433120793));
#123631=CARTESIAN_POINT('Ctrl Pts',(-20.6691708737799,-20.8005034859668,
-3.89828013788936));
#123632=CARTESIAN_POINT('Ctrl Pts',(-21.3357701902385,-18.3253874199006,
-4.02545594457079));
#123633=CARTESIAN_POINT('Ctrl Pts',(-19.6154068412282,-16.4251495041048,
-4.15263175125223));
#123634=CARTESIAN_POINT('Ctrl Pts',(-17.0864074216668,-16.8431400842676,
-4.27980755793366));
#123635=CARTESIAN_POINT('Ctrl Pts',(-16.068971931599,-19.1958787465047,
-4.4069833646151));
#123636=CARTESIAN_POINT('Ctrl Pts',(-17.4965342839917,-21.3248737956469,
-4.53415917129653));
#123637=CARTESIAN_POINT('Ctrl Pts',(-20.0593946250379,-21.2769044144401,
-4.66133497797797));
#123638=CARTESIAN_POINT('Ctrl Pts',(-21.4062876608796,-19.0959795328267,
-4.7885107846594));
#123639=CARTESIAN_POINT('Ctrl Pts',(-20.3015226287422,-16.7829623662223,
-4.91568659134084));
#123640=CARTESIAN_POINT('Ctrl Pts',(-17.7586528761605,-16.4599026029505,
-5.04286239802226));
#123641=CARTESIAN_POINT('Ctrl Pts',(-16.1106035728318,-18.4231875244628,
-5.17003820470371));
#123642=CARTESIAN_POINT('Ctrl Pts',(-16.8693576650841,-20.8716250704767,
-5.29721401138513));
#123643=CARTESIAN_POINT('Ctrl Pts',(-19.3388053668663,-21.5589257596971,
-5.42438981806658));
#123644=CARTESIAN_POINT('Ctrl Pts',(-21.2533816830032,-19.8545338684562,
-5.551565624748));
#123645=CARTESIAN_POINT('Ctrl Pts',(-20.8565816754472,-17.3221231704762,
-5.67874143142944));
#123646=CARTESIAN_POINT('Ctrl Pts',(-18.5124447229449,-16.2850233020193,
-5.80591723811088));
#123647=CARTESIAN_POINT('Ctrl Pts',(-16.3715709858693,-17.6947090227174,
-5.93309304479231));
#123648=CARTESIAN_POINT('Ctrl Pts',(-16.3980792403773,-20.2578811787933,
-6.06026885147374));
#123649=CARTESIAN_POINT('Ctrl Pts',(-18.5676498082457,-21.6229884054533,
-6.18744465815518));
#123650=CARTESIAN_POINT('Ctrl Pts',(-20.8898363521913,-20.5376295503469,
-6.31462046483661));
#123651=CARTESIAN_POINT('Ctrl Pts',(-21.2341768492959,-17.9975539980662,
-6.44179627151804));
#123652=CARTESIAN_POINT('Ctrl Pts',(-19.2847602656477,-16.33312341296,-6.56897207819949));
#123653=CARTESIAN_POINT('Ctrl Pts',(-16.830055322305,-17.0713495506502,
-6.6961478848809));
#123654=CARTESIAN_POINT('Ctrl Pts',(-16.1221014486134,-19.5349557492877,
-6.82332369156236));
#123655=CARTESIAN_POINT('Ctrl Pts',(-17.810402383112,-21.4637362302682,
-6.95049949824377));
#123656=CARTESIAN_POINT('Ctrl Pts',(-20.3460468061722,-21.0881546159098,
-7.07767530492523));
#123657=CARTESIAN_POINT('Ctrl Pts',(-21.4027383394782,-18.7527837261624,
-7.20485111160664));
#123658=CARTESIAN_POINT('Ctrl Pts',(-20.0110280868951,-16.6001814029045,
-7.3320269182881));
#123659=CARTESIAN_POINT('Ctrl Pts',(-17.4477238258878,-16.6052266721572,
-7.45920272496951));
#123660=CARTESIAN_POINT('Ctrl Pts',(-16.0644981193252,-18.7632908125259,
-7.58637853165096));
#123661=CARTESIAN_POINT('Ctrl Pts',(-17.130374700309,-21.0944839197888,
-7.71355433833239));
#123662=CARTESIAN_POINT('Ctrl Pts',(-19.6674779615479,-21.4600810081947,
-7.84073014501382));
#123663=CARTESIAN_POINT('Ctrl Pts',(-21.3481731312431,-19.5246694406454,
-7.96790595169526));
#123664=CARTESIAN_POINT('Ctrl Pts',(-20.630526706906,-17.0638692051782,
-8.09508175837669));
#123665=CARTESIAN_POINT('Ctrl Pts',(-18.1729347407055,-16.3353117833461,
-8.22225756505813));
#123666=CARTESIAN_POINT('Ctrl Pts',(-16.2300853262702,-18.0074033903068,
-8.34943337173957));
#123667=CARTESIAN_POINT('Ctrl Pts',(-16.5844222145103,-20.5461037583834,
-8.47660917842099));
#123668=CARTESIAN_POINT('Ctrl Pts',(-18.910863303093,-21.622312869381,-8.60378498510243));
#123669=CARTESIAN_POINT('Ctrl Pts',(-21.0750432884624,-20.2486756610299,
-8.73096079178387));
#123670=CARTESIAN_POINT('Ctrl Pts',(-21.091461358201,-17.685419014452,-8.8581365984653));
#123671=CARTESIAN_POINT('Ctrl Pts',(-18.9450549523438,-16.2841718092325,
-8.98531240514673));
#123672=CARTESIAN_POINT('Ctrl Pts',(-16.6050187272589,-17.3304913849503,
-9.11248821182817));
#123673=CARTESIAN_POINT('Ctrl Pts',(-16.2181906804335,-19.8644444728012,
-9.2396640185096));
#123674=CARTESIAN_POINT('Ctrl Pts',(-18.1394615355737,-21.561286389548,
-9.36683982519104));
#123675=CARTESIAN_POINT('Ctrl Pts',(-20.6061845306062,-20.8642699944625,
-9.49401563187247));
#123676=CARTESIAN_POINT('Ctrl Pts',(-21.3552944196844,-18.4128645683191,
-9.62119143855391));
#123677=CARTESIAN_POINT('Ctrl Pts',(-19.6995293745825,-16.4560824382241,
-9.74836724523534));
#123678=CARTESIAN_POINT('Ctrl Pts',(-17.1579510558127,-16.7891497569436,
-9.87554305191677));
#123679=CARTESIAN_POINT('Ctrl Pts',(-16.062299822705,-19.1064979320416,
-10.0027188585982));
#123680=CARTESIAN_POINT('Ctrl Pts',(-17.417767677851,-21.2821038437145,
-10.1298946652796));
#123681=CARTESIAN_POINT('Ctrl Pts',(-19.9807969939772,-21.3199841013343,
-10.257070471961));
#123682=CARTESIAN_POINT('Ctrl Pts',(-21.3999674530782,-19.1853859196488,
-10.3842462786425));
#123683=CARTESIAN_POINT('Ctrl Pts',(-20.3732782425814,-16.8366706422493,
-10.5114220853239));
#123684=CARTESIAN_POINT('Ctrl Pts',(-17.8426529895985,-16.4286387584391,
-10.6385978920053));
#123685=CARTESIAN_POINT('Ctrl Pts',(-16.1297832954242,-18.3356341962992,
-10.7657736986868));
#123686=CARTESIAN_POINT('Ctrl Pts',(-16.8061207917803,-20.8081070030786,
-10.8929495053682));
#123687=CARTESIAN_POINT('Ctrl Pts',(-19.2511678039994,-21.5777168375263,
-11.0201253120496));
#123688=CARTESIAN_POINT('Ctrl Pts',(-21.221745455103,-19.9383944439102,
-11.1473011187311));
#123689=CARTESIAN_POINT('Ctrl Pts',(-20.9099710580464,-17.3941163705504,
-11.2744769254125));
#123690=CARTESIAN_POINT('Ctrl Pts',(-18.6018782712276,-16.2790998340474,
-11.401652732094));
#123691=CARTESIAN_POINT('Ctrl Pts',(-16.414998970158,-17.6163033009118,
-11.5288285387754));
#123692=CARTESIAN_POINT('Ctrl Pts',(-16.3556591805319,-20.1789255865028,
-11.6560043454568));
#123693=CARTESIAN_POINT('Ctrl Pts',(-18.4782994762885,-21.6159197980676,
-11.7831801521383));
#123694=CARTESIAN_POINT('Ctrl Pts',(-20.8355291319859,-20.6089329364152,
-11.9103559588197));
#123695=CARTESIAN_POINT('Ctrl Pts',(-21.2647362446946,-18.0818129464581,
-12.0375317655011));
#123696=CARTESIAN_POINT('Ctrl Pts',(-19.372149928102,-16.3530355682261,
-12.1647075721826));
#123697=CARTESIAN_POINT('Ctrl Pts',(-16.8941006605274,-17.0086467462216,
-12.291883378864));
#123698=CARTESIAN_POINT('Ctrl Pts',(-16.1040448398867,-19.4471639164526,
-12.4190591855454));
#123699=CARTESIAN_POINT('Ctrl Pts',(-17.7268096452235,-21.4313989266772,
-12.5462349922269));
#123700=CARTESIAN_POINT('Ctrl Pts',(-20.2736090877839,-21.1409393105282,
-12.6734107989083));
#123701=CARTESIAN_POINT('Ctrl Pts',(-21.4079127512197,-18.8422637378655,
-12.8005866055897));
#123702=CARTESIAN_POINT('Ctrl Pts',(-20.0890674271536,-16.6442643747106,
-12.9277624122712));
#123703=CARTESIAN_POINT('Ctrl Pts',(-17.5270318436439,-16.563469213532,
-13.0549382189526));
#123704=CARTESIAN_POINT('Ctrl Pts',(-16.0723146306984,-18.6740027999979,
-13.182114025634));
#123705=CARTESIAN_POINT('Ctrl Pts',(-17.0595285412618,-21.0395815630135,
-13.3092898323155));
#123706=CARTESIAN_POINT('Ctrl Pts',(-19.5829660857976,-21.4899338118888,
-13.4364656389969));
#123707=CARTESIAN_POINT('Ctrl Pts',(-21.3275299393921,-19.6118893102937,
-13.5636414456783));
#123708=CARTESIAN_POINT('Ctrl Pts',(-20.6926910462166,-17.1284373238537,
-13.6908172523598));
#123709=CARTESIAN_POINT('Ctrl Pts',(-18.2608746882143,-16.3179909097138,
-13.8179930590412));
#123710=CARTESIAN_POINT('Ctrl Pts',(-16.2631214383067,-17.9240843508695,
-13.9451688657226));
#123711=CARTESIAN_POINT('Ctrl Pts',(-16.5322459087333,-20.4732266004621,
-14.0723446724041));
#123712=CARTESIAN_POINT('Ctrl Pts',(-18.8213431016262,-21.6267378621019,
-14.1995204790855));
#123713=CARTESIAN_POINT('Ctrl Pts',(-21.0303084199013,-20.3263431482177,
-14.326696285767));
#123714=CARTESIAN_POINT('Ctrl Pts',(-21.1325532878912,-17.7650738971998,
-14.4538720924484));
#123715=CARTESIAN_POINT('Ctrl Pts',(-19.0342743852475,-16.2927356765588,
-14.5810478991298));
#123716=CARTESIAN_POINT('Ctrl Pts',(-16.6605123712694,-17.2601074201168,
-14.7082237058113));
#123717=CARTESIAN_POINT('Ctrl Pts',(-16.1890465614952,-19.779685595021,
-14.8353995124927));
#123718=CARTESIAN_POINT('Ctrl Pts',(-18.0524175739244,-21.5399136084552,
-14.9625753191741));
#123719=CARTESIAN_POINT('Ctrl Pts',(-20.5410981585017,-20.9258915101652,
-15.0897511258555));
#123720=CARTESIAN_POINT('Ctrl Pts',(-21.3718783438148,-18.5009464648227,
-15.216926932537));
#123721=CARTESIAN_POINT('Ctrl Pts',(-19.7825688738725,-16.4898150424656,
-15.3441027392184));
#123722=CARTESIAN_POINT('Ctrl Pts',(-17.2312625436763,-16.7375854982129,
-15.4712785458999));
#123723=CARTESIAN_POINT('Ctrl Pts',(-16.0586245592516,-19.0169438172852,
-15.5984543525813));
#123724=CARTESIAN_POINT('Ctrl Pts',(-17.3404774891864,-21.2367202148663,
-15.7256301592627));
#123725=CARTESIAN_POINT('Ctrl Pts',(-19.9008008310311,-21.3604076210367,
-15.8528059659442));
#123726=CARTESIAN_POINT('Ctrl Pts',(-21.3906568302317,-19.2745305175414,
-15.9799817726256));
#123727=CARTESIAN_POINT('Ctrl Pts',(-20.4431950784137,-16.8927516827034,
-16.107157579307));
#123728=CARTESIAN_POINT('Ctrl Pts',(-17.9276529267619,-16.40020536762,-16.2343333859885));
#123729=CARTESIAN_POINT('Ctrl Pts',(-16.1518841672621,-18.2487722455082,
-16.3615091926699));
#123730=CARTESIAN_POINT('Ctrl Pts',(-16.7450464201164,-20.7425069409056,
-16.4886849993513));
#123731=CARTESIAN_POINT('Ctrl Pts',(-19.1629501341323,-21.5935626494162,
-16.6158608060327));
#123732=CARTESIAN_POINT('Ctrl Pts',(-21.1873187237296,-20.0211485809561,
-16.7430366127142));
#123733=CARTESIAN_POINT('Ctrl Pts',(-20.9609196544379,-17.4678570483134,
-16.8702124193956));
#123734=CARTESIAN_POINT('Ctrl Pts',(-18.6914600204213,-16.276174557543,
-16.9973882260771));
#123735=CARTESIAN_POINT('Ctrl Pts',(-16.4610281773391,-17.5393958297695,
-17.1245640327585));
#123736=CARTESIAN_POINT('Ctrl Pts',(-16.3159069050066,-20.0985937520796,
-17.2517398394399));
#123737=CARTESIAN_POINT('Ctrl Pts',(-18.3892359635466,-21.6058630724912,
-17.3789156461214));
#123738=CARTESIAN_POINT('Ctrl Pts',(-20.7788646270633,-20.6783777412105,
-17.5060914528028));
#123739=CARTESIAN_POINT('Ctrl Pts',(-21.2924569138617,-18.1670479834574,
-17.6332672594842));
#123740=CARTESIAN_POINT('Ctrl Pts',(-19.458823777937,-16.3758629812631,
-17.7604430661657));
#123741=CARTESIAN_POINT('Ctrl Pts',(-16.9602098133921,-16.9481238006687,
-17.8876188728471));
#123742=CARTESIAN_POINT('Ctrl Pts',(-16.0889382512251,-19.3588166583677,
-18.0147946795285));
#123743=CARTESIAN_POINT('Ctrl Pts',(-17.6443466725109,-21.3962804819219,
-18.14197048621));
#123744=CARTESIAN_POINT('Ctrl Pts',(-20.1994443902567,-21.1912686724342,
-18.2691462928914));
#123745=CARTESIAN_POINT('Ctrl Pts',(-21.4100878356756,-18.9318668407438,
-18.3963220995729));
#123746=CARTESIAN_POINT('Ctrl Pts',(-20.1655867886111,-16.6909359329365,
-18.5234979062543));
#123747=CARTESIAN_POINT('Ctrl Pts',(-17.607693717282,-16.5243909694468,
-18.6506737129357));
#123748=CARTESIAN_POINT('Ctrl Pts',(-16.0831167539157,-18.5850266165988,
-18.7778495196171));
#123749=CARTESIAN_POINT('Ctrl Pts',(-16.9905606364213,-20.9823375670122,
-18.9050253262986));
#123750=CARTESIAN_POINT('Ctrl Pts',(-19.4975019250372,-21.5169398148659,
-19.03220113298));
#123751=CARTESIAN_POINT('Ctrl Pts',(-21.3039775855559,-19.6983689841434,
-19.1593769396615));
#123752=CARTESIAN_POINT('Ctrl Pts',(-20.7526583224132,-17.1950509287168,
-19.2865527463429));
#123753=CARTESIAN_POINT('Ctrl Pts',(-18.3493453399679,-16.3036246104209,
-19.4137285530243));
#123754=CARTESIAN_POINT('Ctrl Pts',(-16.2989291348091,-17.8419183107137,
-19.5409043597057));
#123755=CARTESIAN_POINT('Ctrl Pts',(-16.4825393088626,-20.3986431089516,
-19.6680801663872));
#123756=CARTESIAN_POINT('Ctrl Pts',(-18.7317249295881,-21.6281625520724,
-19.7952559730686));
#123757=CARTESIAN_POINT('Ctrl Pts',(-20.9829977785724,-20.402469131249,
-19.9224317797501));
#123758=CARTESIAN_POINT('Ctrl Pts',(-21.1709547689763,-17.8460599692811,
-20.0496075864315));
#123759=CARTESIAN_POINT('Ctrl Pts',(-19.1231569849638,-16.3042827972216,
-20.1767833931129));
#123760=CARTESIAN_POINT('Ctrl Pts',(-16.7183318756798,-17.191620562574,
-20.3039591997943));
#123761=CARTESIAN_POINT('Ctrl Pts',(-16.1627570587368,-19.6939996284889,
-20.4311350064758));
#123762=CARTESIAN_POINT('Ctrl Pts',(-17.9661382538539,-21.5156354105067,
-20.5583108131572));
#123763=CARTESIAN_POINT('Ctrl Pts',(-20.4739845514727,-20.9853038346024,
-20.6854866198387));
#123764=CARTESIAN_POINT('Ctrl Pts',(-21.3855037715295,-18.5895248239564,
-20.8126624265201));
#123765=CARTESIAN_POINT('Ctrl Pts',(-19.8644314016694,-16.5263277520078,
-20.9398382332015));
#123766=CARTESIAN_POINT('Ctrl Pts',(-17.3062611778333,-16.6884699406521,
-21.067014039883));
#123767=CARTESIAN_POINT('Ctrl Pts',(-16.0579473234008,-18.9273846894854,
-21.1941898465644));
#123768=CARTESIAN_POINT('Ctrl Pts',(-17.2647560806485,-21.1886431148375,
-21.3213656532458));
#123769=CARTESIAN_POINT('Ctrl Pts',(-19.8194849413283,-21.3983814848332,
-21.4485414599273));
#123770=CARTESIAN_POINT('Ctrl Pts',(-21.3783873758939,-19.3628277961746,
-21.5757172666087));
#123771=CARTESIAN_POINT('Ctrl Pts',(-20.5111531531137,-16.9520807626706,
-21.7028930732902));
#123772=CARTESIAN_POINT('Ctrl Pts',(-18.0136452314969,-16.3728012940309,
-21.8300688799716));
#123773=CARTESIAN_POINT('Ctrl Pts',(-16.1763689660104,-18.1667340430625,
-21.9572633429927));
#123774=CARTESIAN_POINT('Ctrl Pts',(-16.5172187855734,-19.8331819102064,
-22.0420658704533));
#123775=CARTESIAN_POINT('Ctrl Pts',(-17.0028271735668,-20.4098093075325,
-22.0844764623534));
#123776=CARTESIAN_POINT('Ctrl Pts',(-19.2802416597141,-20.9933733729761,
0.257964067486649));
#123777=CARTESIAN_POINT('Ctrl Pts',(-19.9599077040175,-20.8115046795727,
0.215572131926171));
#123778=CARTESIAN_POINT('Ctrl Pts',(-21.1114426467799,-19.7184754707294,
0.130788260805215));
#123779=CARTESIAN_POINT('Ctrl Pts',(-20.6647168313355,-17.3632029388733,
0.00361245412378029));
#123780=CARTESIAN_POINT('Ctrl Pts',(-18.4433885306129,-16.4708798215613,
-0.123563352557654));
#123781=CARTESIAN_POINT('Ctrl Pts',(-16.4903434967449,-17.8521961917666,
-0.250739159239088));
#123782=CARTESIAN_POINT('Ctrl Pts',(-16.5948541842955,-20.2438677216565,
-0.377914965920522));
#123783=CARTESIAN_POINT('Ctrl Pts',(-18.6623442009214,-21.4496298079404,
-0.505090772601956));
#123784=CARTESIAN_POINT('Ctrl Pts',(-20.7953426306735,-20.3643352377974,
-0.632266579283392));
#123785=CARTESIAN_POINT('Ctrl Pts',(-21.0373071996992,-17.9831220108,-0.759442385964825));
#123786=CARTESIAN_POINT('Ctrl Pts',(-19.1660680589383,-16.4908921587843,
-0.886618192646261));
#123787=CARTESIAN_POINT('Ctrl Pts',(-16.8984656329369,-17.2565251572569,
-1.0137939993277));
#123788=CARTESIAN_POINT('Ctrl Pts',(-16.3148352767375,-19.5776774778398,
-1.14096980600913));
#123789=CARTESIAN_POINT('Ctrl Pts',(-17.9506471159836,-21.3247958511667,
-1.26814561269057));
#123790=CARTESIAN_POINT('Ctrl Pts',(-20.3051320841986,-20.8950284114407,
-1.395321419372));
#123791=CARTESIAN_POINT('Ctrl Pts',(-21.2182032274825,-18.6826493129518,
-1.52249722605343));
#123792=CARTESIAN_POINT('Ctrl Pts',(-19.8521708785292,-16.7173846668031,
-1.64967303273487));
#123793=CARTESIAN_POINT('Ctrl Pts',(-17.4602867822325,-16.8022398991988,
-1.7768488394163));
#123794=CARTESIAN_POINT('Ctrl Pts',(-16.2369551795592,-18.8593671107158,
-1.90402464609774));
#123795=CARTESIAN_POINT('Ctrl Pts',(-17.3045073858597,-21.0014789809986,
-2.03120045277917));
#123796=CARTESIAN_POINT('Ctrl Pts',(-19.6835302529274,-21.2633212301712,
-2.15837625946061));
#123797=CARTESIAN_POINT('Ctrl Pts',(-21.1914180933035,-19.4046696353217,
-2.28555206614204));
#123798=CARTESIAN_POINT('Ctrl Pts',(-20.4447773338319,-17.1307217833394,
-2.41272787282348));
#123799=CARTESIAN_POINT('Ctrl Pts',(-18.1286045657439,-16.5276836344422,
-2.53990367950491));
#123800=CARTESIAN_POINT('Ctrl Pts',(-16.3678445270935,-18.1488052909833,
-2.66707948618633));
#123801=CARTESIAN_POINT('Ctrl Pts',(-16.7778852779924,-20.5068082359283,
-2.79425529286778));
#123802=CARTESIAN_POINT('Ctrl Pts',(-18.9825398744333,-21.4383711294077,
-2.92143109954921));
#123803=CARTESIAN_POINT('Ctrl Pts',(-20.9591745631026,-20.0888428318423,
-3.04860690623065));
#123804=CARTESIAN_POINT('Ctrl Pts',(-20.8943496995691,-17.6963317972172,
-3.17578271291207));
#123805=CARTESIAN_POINT('Ctrl Pts',(-18.847538073347,-16.4558184027074,
-3.30295851959352));
#123806=CARTESIAN_POINT('Ctrl Pts',(-16.6965623116711,-17.5053966934078,
-3.43013432627495));
#123807=CARTESIAN_POINT('Ctrl Pts',(-16.4148091714573,-19.8821437314771,
-3.55731013295638));
#123808=CARTESIAN_POINT('Ctrl Pts',(-18.2607696711808,-21.4055416272001,
-3.68448593963782));
#123809=CARTESIAN_POINT('Ctrl Pts',(-20.5408896256266,-20.6779673639072,
-3.81166174631925));
#123810=CARTESIAN_POINT('Ctrl Pts',(-21.163300496769,-18.3669251698599,
-3.93883755300069));
#123811=CARTESIAN_POINT('Ctrl Pts',(-19.5569789415241,-16.5926528186193,
-4.06601335968212));
#123812=CARTESIAN_POINT('Ctrl Pts',(-17.1956252872621,-16.9829350686982,
-4.19318916636356));
#123813=CARTESIAN_POINT('Ctrl Pts',(-16.2456349496354,-19.1797121792916,
-4.32036497304499));
#123814=CARTESIAN_POINT('Ctrl Pts',(-17.5785651003642,-21.1675774987978,
-4.44754077972642));
#123815=CARTESIAN_POINT('Ctrl Pts',(-19.9715350571314,-21.1227879774049,
-4.57471658640786));
#123816=CARTESIAN_POINT('Ctrl Pts',(-21.2291434090686,-19.0864352210401,
-4.70189239308929));
#123817=CARTESIAN_POINT('Ctrl Pts',(-20.197612549251,-16.9267464933619,
-4.82906819977073));
#123818=CARTESIAN_POINT('Ctrl Pts',(-17.8233080175354,-16.6251021566151,
-4.95624400645216));
#123819=CARTESIAN_POINT('Ctrl Pts',(-16.284506855812,-18.4582421676058,
-5.0834198131336));
#123820=CARTESIAN_POINT('Ctrl Pts',(-16.9929636211903,-20.7443743437509,
-5.21059561981502));
#123821=CARTESIAN_POINT('Ctrl Pts',(-19.298713203222,-21.3861143068026,
-5.33777142649647));
#123822=CARTESIAN_POINT('Ctrl Pts',(-21.0863734713516,-19.7947054715354,
-5.4649472331779));
#123823=CARTESIAN_POINT('Ctrl Pts',(-20.7158770842802,-17.4301666703347,
-5.59212303985933));
#123824=CARTESIAN_POINT('Ctrl Pts',(-18.5271314815462,-16.4618154934729,
-5.71929884654077));
#123825=CARTESIAN_POINT('Ctrl Pts',(-16.5281749047854,-17.7780540430683,
-5.8464746532222));
#123826=CARTESIAN_POINT('Ctrl Pts',(-16.552925943938,-20.171315144845,-5.97365045990364));
#123827=CARTESIAN_POINT('Ctrl Pts',(-18.5786770568045,-21.4459302804593,
-6.10082626658507));
#123828=CARTESIAN_POINT('Ctrl Pts',(-20.7469273296236,-20.4325191745226,
-6.22800207326651));
#123829=CARTESIAN_POINT('Ctrl Pts',(-21.0684417138734,-18.0608236173447,
-6.35517787994794));
#123830=CARTESIAN_POINT('Ctrl Pts',(-19.2482507174378,-16.5067270786087,
-6.48235368662938));
#123831=CARTESIAN_POINT('Ctrl Pts',(-16.9562666057522,-17.1960166744951,
-6.6095294933108));
#123832=CARTESIAN_POINT('Ctrl Pts',(-16.2952425447106,-19.4963119829154,
-6.73670529999224));
#123833=CARTESIAN_POINT('Ctrl Pts',(-17.8716270825383,-21.2972348308226,
-6.86388110667369));
#123834=CARTESIAN_POINT('Ctrl Pts',(-20.2391852472374,-20.94655028314,-6.9910569133551));
#123835=CARTESIAN_POINT('Ctrl Pts',(-21.2258293699287,-18.7659896464285,
-7.11823272003656));
#123836=CARTESIAN_POINT('Ctrl Pts',(-19.9263747060834,-16.7560819640143,
-7.24540852671797));
#123837=CARTESIAN_POINT('Ctrl Pts',(-17.5329902565274,-16.7607927855726,
-7.37258433339943));
#123838=CARTESIAN_POINT('Ctrl Pts',(-16.2414577035358,-18.7758002247102,
-7.49976014008084));
#123839=CARTESIAN_POINT('Ctrl Pts',(-17.2366780029277,-20.9524600214847,
-7.62693594676229));
#123840=CARTESIAN_POINT('Ctrl Pts',(-19.6055983003493,-21.293821911099,
-7.75411175344372));
#123841=CARTESIAN_POINT('Ctrl Pts',(-21.1748812546918,-19.48670754714,-7.88128756012516));
#123842=CARTESIAN_POINT('Ctrl Pts',(-20.5048071560311,-17.1890321963735,
-8.00846336680658));
#123843=CARTESIAN_POINT('Ctrl Pts',(-18.2101274003992,-16.5087703833118,
-8.13563917348801));
#123844=CARTESIAN_POINT('Ctrl Pts',(-16.3960682397005,-18.0700200996293,
-8.26281498016946));
#123845=CARTESIAN_POINT('Ctrl Pts',(-16.7269163606663,-20.4404316326905,
-8.38999078685089));
#123846=CARTESIAN_POINT('Ctrl Pts',(-18.8991391470608,-21.4452995252443,
-8.51716659353233));
#123847=CARTESIAN_POINT('Ctrl Pts',(-20.9198570157183,-20.1627198550076,
-8.64434240021374));
#123848=CARTESIAN_POINT('Ctrl Pts',(-20.9351867420414,-17.7693798635505,
-8.77151820689519));
#123849=CARTESIAN_POINT('Ctrl Pts',(-18.9310642535986,-16.4610204456021,
-8.89869401357662));
#123850=CARTESIAN_POINT('Ctrl Pts',(-16.7461475436661,-17.4379801611861,
-9.02586982025806));
#123851=CARTESIAN_POINT('Ctrl Pts',(-16.3849620823817,-19.8039591082128,
-9.15304562693949));
#123852=CARTESIAN_POINT('Ctrl Pts',(-18.1788731127761,-21.3883184520001,
-9.28022143362092));
#123853=CARTESIAN_POINT('Ctrl Pts',(-20.4820786071378,-20.7375068310543,
-9.40739724030236));
#123854=CARTESIAN_POINT('Ctrl Pts',(-21.1815304774453,-18.4486035136685,
-9.53457304698381));
#123855=CARTESIAN_POINT('Ctrl Pts',(-19.6355250455705,-16.6215352281822,
-9.66174885366522));
#123856=CARTESIAN_POINT('Ctrl Pts',(-17.2624263393396,-16.932523725882,
-9.78892466034668));
#123857=CARTESIAN_POINT('Ctrl Pts',(-16.2394051306023,-19.0962563622516,
-9.91610046702808));
#123858=CARTESIAN_POINT('Ctrl Pts',(-17.5050198825181,-21.1276427398149,
-10.0432762737096));
#123859=CARTESIAN_POINT('Ctrl Pts',(-19.8981476131147,-21.1630119392157,
-10.170452080391));
#123860=CARTESIAN_POINT('Ctrl Pts',(-21.2232421638282,-19.1699149152638,
-10.2976278870724));
#123861=CARTESIAN_POINT('Ctrl Pts',(-20.2646115290223,-16.9768944818824,
-10.4248036937539));
#123862=CARTESIAN_POINT('Ctrl Pts',(-17.901739816804,-16.5959107725,-10.5519795004353));
#123863=CARTESIAN_POINT('Ctrl Pts',(-16.3024151667752,-18.3764926939591,
-10.6791553071167));
#123864=CARTESIAN_POINT('Ctrl Pts',(-16.9339186800547,-20.6850668486988,
-10.8063311137982));
#123865=CARTESIAN_POINT('Ctrl Pts',(-19.2168850787369,-21.4036597360172,
-10.9335069204796));
#123866=CARTESIAN_POINT('Ctrl Pts',(-21.0568343889061,-19.8730069827043,
-11.0606827271611));
#123867=CARTESIAN_POINT('Ctrl Pts',(-20.7657273186155,-17.4973874869004,
-11.1878585338425));
#123868=CARTESIAN_POINT('Ctrl Pts',(-18.6106365367144,-16.4562846884308,
-11.3150343405239));
#123869=CARTESIAN_POINT('Ctrl Pts',(-16.5687240755777,-17.7048457867641,
-11.4422101472054));
#123870=CARTESIAN_POINT('Ctrl Pts',(-16.5133178829179,-20.0975934686209,
-11.5693859538868));
#123871=CARTESIAN_POINT('Ctrl Pts',(-18.4952497016042,-21.4393302465677,
-11.6965617605682));
#123872=CARTESIAN_POINT('Ctrl Pts',(-20.6962201005539,-20.4990959044147,
-11.8237375672497));
#123873=CARTESIAN_POINT('Ctrl Pts',(-21.09697534636,-18.1394970935624,-11.9509133739311));
#123874=CARTESIAN_POINT('Ctrl Pts',(-19.3298473746713,-16.5253192697488,
-12.0780891806125));
#123875=CARTESIAN_POINT('Ctrl Pts',(-17.0160664191804,-17.1374703991481,
-12.205264987294));
#123876=CARTESIAN_POINT('Ctrl Pts',(-16.2783828971083,-19.4143398149205,
-12.3324407939754));
#123877=CARTESIAN_POINT('Ctrl Pts',(-17.7935756541529,-21.2670411465485,
-12.4596166006568));
#123878=CARTESIAN_POINT('Ctrl Pts',(-20.1715493791944,-20.9958359138768,
-12.5867924073383));
#123879=CARTESIAN_POINT('Ctrl Pts',(-21.2306607732021,-18.8495380849864,
-12.7139682140197));
#123880=CARTESIAN_POINT('Ctrl Pts',(-19.9992408680408,-16.7972427036174,
-12.8411440207011));
#123881=CARTESIAN_POINT('Ctrl Pts',(-17.6070409961567,-16.7218034023586,
-12.9683198273826));
#123882=CARTESIAN_POINT('Ctrl Pts',(-16.2487560633345,-18.6924310578239,
-13.095495634064));
#123883=CARTESIAN_POINT('Ctrl Pts',(-17.1705281907678,-20.9011971070702,
-13.2226714407454));
#123884=CARTESIAN_POINT('Ctrl Pts',(-19.526688663167,-21.3216957913963,
-13.3498472474269));
#123885=CARTESIAN_POINT('Ctrl Pts',(-21.1556064869176,-19.5681456670245,
-13.4770230541083));
#123886=CARTESIAN_POINT('Ctrl Pts',(-20.5628506607707,-17.2493201354707,
-13.6041988607897));
#123887=CARTESIAN_POINT('Ctrl Pts',(-18.2922378646403,-16.4925976993917,
-13.7313746674712));
#123888=CARTESIAN_POINT('Ctrl Pts',(-16.426914408852,-17.9922242263985,
-13.8585504741526));
#123889=CARTESIAN_POINT('Ctrl Pts',(-16.6781987890609,-20.3723854552819,
-13.985726280834));
#123890=CARTESIAN_POINT('Ctrl Pts',(-18.8155531828929,-21.449431188008,
-14.1129020875155));
#123891=CARTESIAN_POINT('Ctrl Pts',(-20.878087593182,-20.2352388137978,
-14.2400778941968));
#123892=CARTESIAN_POINT('Ctrl Pts',(-20.973554713811,-17.8437544747116,
-14.3672537008784));
#123893=CARTESIAN_POINT('Ctrl Pts',(-19.0143693869603,-16.4690166196025,
-14.4944295075598));
#123894=CARTESIAN_POINT('Ctrl Pts',(-16.7979625492603,-17.372261904679,
-14.6216053142412));
#123895=CARTESIAN_POINT('Ctrl Pts',(-16.3577499085777,-19.7248188426085,
-14.7487811209226));
#123896=CARTESIAN_POINT('Ctrl Pts',(-18.097599240061,-21.3683624589916,
-14.8759569276041));
#123897=CARTESIAN_POINT('Ctrl Pts',(-20.4213067693024,-20.7950434956184,
-15.0031327342855));
#123898=CARTESIAN_POINT('Ctrl Pts',(-21.1970150637779,-18.5308465171956,
-15.130308540967));
#123899=CARTESIAN_POINT('Ctrl Pts',(-19.7130599091926,-16.6530317195128,
-15.2574843476484));
#123900=CARTESIAN_POINT('Ctrl Pts',(-17.3308780552345,-16.884377629113,
-15.3846601543298));
#123901=CARTESIAN_POINT('Ctrl Pts',(-16.2359734980291,-19.0126387328847,
-15.5118359610112));
#123902=CARTESIAN_POINT('Ctrl Pts',(-17.4328532113714,-21.0852675628988,
-15.6390117676927));
#123903=CARTESIAN_POINT('Ctrl Pts',(-19.823454345003,-21.2007558094709,
-15.7661875743741));
#123904=CARTESIAN_POINT('Ctrl Pts',(-21.2145487362569,-19.2531501743798,
-15.8933633810556));
#123905=CARTESIAN_POINT('Ctrl Pts',(-20.3298936222131,-17.0292579457831,
-16.020539187737));
#123906=CARTESIAN_POINT('Ctrl Pts',(-17.9811051621181,-16.5693622130996,
-16.1477149944184));
#123907=CARTESIAN_POINT('Ctrl Pts',(-16.3230509858558,-18.295388766718,
-16.2748908010999));
#123908=CARTESIAN_POINT('Ctrl Pts',(-16.8768928896987,-20.6238153729833,
-16.4020666077813));
#123909=CARTESIAN_POINT('Ctrl Pts',(-19.1345153021762,-21.418455139101,
-16.5292424144627));
#123910=CARTESIAN_POINT('Ctrl Pts',(-21.0246897836904,-19.9502754005642,
-16.6564182211442));
#123911=CARTESIAN_POINT('Ctrl Pts',(-20.8132985649108,-17.5662399419689,
-16.7835940278256));
#123912=CARTESIAN_POINT('Ctrl Pts',(-18.6942799686495,-16.4535533266478,
-16.910769834507));
#123913=CARTESIAN_POINT('Ctrl Pts',(-16.6117020358488,-17.6330364630381,
-17.0379456411885));
#123914=CARTESIAN_POINT('Ctrl Pts',(-16.4762007604896,-20.0225867804811,
-17.1651214478699));
#123915=CARTESIAN_POINT('Ctrl Pts',(-18.4120901525558,-21.4299401749425,
-17.2922972545513));
#123916=CARTESIAN_POINT('Ctrl Pts',(-20.6433118496738,-20.563937257206,
-17.4194730612328));
#123917=CARTESIAN_POINT('Ctrl Pts',(-21.1228584299742,-18.2190819540937,
-17.5466488679142));
#123918=CARTESIAN_POINT('Ctrl Pts',(-19.4107756700491,-16.5466334680738,
-17.6738246745956));
#123919=CARTESIAN_POINT('Ctrl Pts',(-17.0777932382892,-17.0809594812165,
-17.8010004812771));
#123920=CARTESIAN_POINT('Ctrl Pts',(-16.2642777146144,-19.3318490404626,
-17.9281762879585));
#123921=CARTESIAN_POINT('Ctrl Pts',(-17.7165790995274,-21.2342506811916,
-18.05535209464));
#123922=CARTESIAN_POINT('Ctrl Pts',(-20.1023010123624,-21.0428289743473,
-18.1825279013214));
#123923=CARTESIAN_POINT('Ctrl Pts',(-21.2326916726909,-18.9332014550839,
-18.3097037080028));
#123924=CARTESIAN_POINT('Ctrl Pts',(-20.0706878096263,-16.8408204338905,
-18.4368795146842));
#123925=CARTESIAN_POINT('Ctrl Pts',(-17.6823558454215,-16.6853156302542,
-18.5640553213657));
#123926=CARTESIAN_POINT('Ctrl Pts',(-16.2588421206643,-18.6093530491115,
-18.6912311280471));
#123927=CARTESIAN_POINT('Ctrl Pts',(-17.1061321245363,-20.8477477792071,
-18.8184069347286));
#123928=CARTESIAN_POINT('Ctrl Pts',(-19.4468898673433,-21.3469115835881,
-18.94558274141));
#123929=CARTESIAN_POINT('Ctrl Pts',(-21.1336154036588,-19.6488926582199,
-19.0727585480914));
#123930=CARTESIAN_POINT('Ctrl Pts',(-20.6188427443147,-17.3115179667752,
-19.1999343547728));
#123931=CARTESIAN_POINT('Ctrl Pts',(-18.3748438530787,-16.4791837329545,
-19.3271101614543));
#123932=CARTESIAN_POINT('Ctrl Pts',(-16.4603484358955,-17.9155049208591,
-19.4542859681357));
#123933=CARTESIAN_POINT('Ctrl Pts',(-16.6317872081259,-20.302746056054,
-19.5814617748171));
#123934=CARTESIAN_POINT('Ctrl Pts',(-18.7318757425608,-21.4507614361853,
-19.7086375814986));
#123935=CARTESIAN_POINT('Ctrl Pts',(-20.8339131442188,-20.3063184537634,
-19.83581338818));
#123936=CARTESIAN_POINT('Ctrl Pts',(-21.0094105851045,-17.9193720315106,
-19.9629891948615));
#123937=CARTESIAN_POINT('Ctrl Pts',(-19.0973600155928,-16.4797982889704,
-20.0901650015429));
#123938=CARTESIAN_POINT('Ctrl Pts',(-16.8519492354458,-17.3083149974252,
-20.2173408082243));
#123939=CARTESIAN_POINT('Ctrl Pts',(-16.3332031202602,-19.6448129443766,
-20.3445166149058));
#123940=CARTESIAN_POINT('Ctrl Pts',(-18.01703932132,-21.3456936473654,-20.4716924215872));
#123941=CARTESIAN_POINT('Ctrl Pts',(-20.358642080658,-20.8505174148026,
-20.5988682282686));
#123942=CARTESIAN_POINT('Ctrl Pts',(-21.2097372705433,-18.6135530731602,
-20.72604403495));
#123943=CARTESIAN_POINT('Ctrl Pts',(-19.7894958220145,-16.6871240247294,
-20.8532198416315));
#123944=CARTESIAN_POINT('Ctrl Pts',(-17.4009050775665,-16.8385179106685,
-20.9803956483129));
#123945=CARTESIAN_POINT('Ctrl Pts',(-16.2353411557127,-18.9290164227857,
-21.1075714549944));
#123946=CARTESIAN_POINT('Ctrl Pts',(-17.3621513269132,-21.0403774632962,
-21.2347472616758));
#123947=CARTESIAN_POINT('Ctrl Pts',(-19.7475288339831,-21.2362124099542,
-21.3619230683572));
#123948=CARTESIAN_POINT('Ctrl Pts',(-21.2030926162545,-19.335594282492,
-21.4890988750387));
#123949=CARTESIAN_POINT('Ctrl Pts',(-20.3933467993028,-17.0846541387204,
-21.6162746817201));
#123950=CARTESIAN_POINT('Ctrl Pts',(-18.0613970915878,-16.5437747381437,
-21.7434504884015));
#123951=CARTESIAN_POINT('Ctrl Pts',(-16.3459127028459,-18.2187888246082,
-21.8706449514226));
#123952=CARTESIAN_POINT('Ctrl Pts',(-16.6641678043512,-19.7747689210369,
-21.9554474788832));
#123953=CARTESIAN_POINT('Ctrl Pts',(-17.117585520725,-20.3131720544228,
-21.9978580707833));
#123954=CARTESIAN_POINT('Ctrl Pts',(-19.3957372685685,-21.4249949024184,
1.39406715338186E-15));
#123955=CARTESIAN_POINT('Ctrl Pts',(-19.4773891020297,-21.3954306668132,
-2.3809056499643E-15));
#123956=CARTESIAN_POINT('Ctrl Pts',(-19.5571492231821,-21.3614659991419,
-1.69827097432457E-14));
#123957=CARTESIAN_POINT('Ctrl Pts',(-19.6348156046203,-21.3234187284543,
-1.60947644101128E-14));
#123958=CARTESIAN_POINT('Ctrl Pts',(-19.7143272588125,-21.2844674940355,
-1.51857224158522E-14));
#123959=CARTESIAN_POINT('Ctrl Pts',(-19.791645221547,-21.2412367046734,
-5.29650342682161E-15));
#123960=CARTESIAN_POINT('Ctrl Pts',(-19.8665232792573,-21.1940209467373,
-3.49026363366534E-15));
#123961=CARTESIAN_POINT('Ctrl Pts',(-19.9365886939582,-21.1498398907462,
-1.80011642596993E-15));
#123962=CARTESIAN_POINT('Ctrl Pts',(-20.0045179028423,-21.1021686855571,
-2.11652109659911E-15));
#123963=CARTESIAN_POINT('Ctrl Pts',(-20.0700783470716,-21.0512211850772,
1.8249290967276E-14));
#123964=CARTESIAN_POINT('Ctrl Pts',(-20.0997467345518,-21.0281656642803,
2.73184124025687E-14));
#123965=CARTESIAN_POINT('Ctrl Pts',(-20.128929580841,-21.0044388940273,
-8.16471876178969E-16));
#123966=CARTESIAN_POINT('Ctrl Pts',(-20.1576029444589,-20.9800594108908,
-2.27595720048157E-15));
#123967=CARTESIAN_POINT('Ctrl Pts',(-20.1753081557669,-20.9650055823179,
-2.81404609490192E-15));
#123968=CARTESIAN_POINT('Ctrl Pts',(-20.1928190804462,-20.9497028729833,
1.46191299131089E-14));
#123969=CARTESIAN_POINT('Ctrl Pts',(-20.2101297684373,-20.9341555341053,
1.78954073781767E-14));
#123970=CARTESIAN_POINT('Ctrl Pts',(-20.2222918053998,-20.923232380144,
1.99869058837013E-14));
#123971=CARTESIAN_POINT('Ctrl Pts',(-20.2343567785502,-20.9121866751007,
2.10812009255155E-14));
#123972=CARTESIAN_POINT('Ctrl Pts',(-20.2463057260566,-20.9010359825867,
1.90611415540332E-14));
#123973=CARTESIAN_POINT('Ctrl Pts',(-20.3097375112913,-20.8418417872492,
8.08726206506259E-15));
#123974=CARTESIAN_POINT('Ctrl Pts',(-20.3700069578684,-20.7796002467127,
1.56207924856702E-14));
#123975=CARTESIAN_POINT('Ctrl Pts',(-20.4268835059677,-20.7145895545046,
1.22124532708767E-15));
#123976=CARTESIAN_POINT('Ctrl Pts',(-20.4830376461181,-20.6504045847144,
-1.29954083951569E-14));
#123977=CARTESIAN_POINT('Ctrl Pts',(-20.5358849804727,-20.5835195230904,
3.31732538375231E-14));
#123978=CARTESIAN_POINT('Ctrl Pts',(-20.5851611052576,-20.5141759583256,
1.8623991238087E-14));
#123979=CARTESIAN_POINT('Ctrl Pts',(-20.6305983443472,-20.4502346450567,
5.20819756122576E-15));
#123980=CARTESIAN_POINT('Ctrl Pts',(-20.6729990002148,-20.3842022515032,
1.20148051242741E-14));
#123981=CARTESIAN_POINT('Ctrl Pts',(-20.7121180817081,-20.3162569684087,
1.55847557081756E-14));
#123982=CARTESIAN_POINT('Ctrl Pts',(-20.7284901400346,-20.2878206121505,
1.73076904422733E-14));
#123983=CARTESIAN_POINT('Ctrl Pts',(-20.7442869378835,-20.2590491139325,
1.78194106763539E-15));
#123984=CARTESIAN_POINT('Ctrl Pts',(-20.7594884026036,-20.2299553026624,
-7.7715611723761E-16));
#123985=CARTESIAN_POINT('Ctrl Pts',(-20.7693451022676,-20.2110907415789,
-2.78913582753658E-15));
#123986=CARTESIAN_POINT('Ctrl Pts',(-20.7789514808442,-20.1920906691223,
5.3858075104116E-15));
#123987=CARTESIAN_POINT('Ctrl Pts',(-20.7883017662921,-20.1729585792041,
1.33226762955019E-14));
#123988=CARTESIAN_POINT('Ctrl Pts',(-20.7942277139279,-20.1608331993265,
1.81940072510115E-14));
#123989=CARTESIAN_POINT('Ctrl Pts',(-20.8000469683619,-20.1486625665028,
-1.84110758617763E-14));
#123990=CARTESIAN_POINT('Ctrl Pts',(-20.8057568610096,-20.1364512427194,
-1.45439216225896E-14));
#123991=CARTESIAN_POINT('Ctrl Pts',(-20.8408823973353,-20.0613308641761,
8.50303143961268E-15));
#123992=CARTESIAN_POINT('Ctrl Pts',(-20.8718944952827,-19.9846287385395,
-1.36466997584689E-15));
#123993=CARTESIAN_POINT('Ctrl Pts',(-20.8985463569486,-19.9065734343537,
8.02136135291676E-15));
#123994=CARTESIAN_POINT('Ctrl Pts',(-20.9251982186144,-19.8285181301678,
1.71371673297255E-14));
#123995=CARTESIAN_POINT('Ctrl Pts',(-20.9474903161071,-19.7491089176507,
2.28815957419719E-14));
#123996=CARTESIAN_POINT('Ctrl Pts',(-20.9651215428786,-19.6685651028304,
1.17683640610267E-14));
#123997=CARTESIAN_POINT('Ctrl Pts',(-20.9829460124324,-19.5871385070737,
3.68731748262102E-16));
#123998=CARTESIAN_POINT('Ctrl Pts',(-20.9960061448808,-19.5045510760419,
8.47281867687301E-15));
#123999=CARTESIAN_POINT('Ctrl Pts',(-21.0043775994437,-19.4211942605515,
5.24580379135386E-15));
#124000=CARTESIAN_POINT('Ctrl Pts',(-21.0078360662703,-19.3867573799617,
3.88824530893464E-15));
#124001=CARTESIAN_POINT('Ctrl Pts',(-21.0104937056419,-19.3521893421996,
-6.81493208789715E-15));
#124002=CARTESIAN_POINT('Ctrl Pts',(-21.0123534306943,-19.3175186761032,
-9.90874049477952E-15));
#124003=CARTESIAN_POINT('Ctrl Pts',(-21.0130853886539,-19.3038728578793,
-1.11360150531808E-14));
#124004=CARTESIAN_POINT('Ctrl Pts',(-21.0136937288726,-19.2902091507495,
-9.58524568179392E-15));
#124005=CARTESIAN_POINT('Ctrl Pts',(-21.0141781582269,-19.2765469516024,
-8.40993941153556E-15));
#124006=CARTESIAN_POINT('Ctrl Pts',(-21.0170629175674,-19.1951890482203,
2.39772407460705E-16));
#124007=CARTESIAN_POINT('Ctrl Pts',(-21.0155663596031,-19.1137544906502,
-4.57265169201993E-15));
#124008=CARTESIAN_POINT('Ctrl Pts',(-21.0098211098971,-19.032600466024,
-7.49400541621981E-15));
#124009=CARTESIAN_POINT('Ctrl Pts',(-21.0040551996084,-18.9511546021348,
-1.04258646664422E-14));
#124010=CARTESIAN_POINT('Ctrl Pts',(-20.9940096109022,-18.8699902747511,
-7.23578815300704E-16));
#124011=CARTESIAN_POINT('Ctrl Pts',(-20.9797677234152,-18.7894801122778,
-9.63118473862323E-15));
#124012=CARTESIAN_POINT('Ctrl Pts',(-20.9656475490784,-18.7096580008453,
-1.84626650234184E-14));
#124013=CARTESIAN_POINT('Ctrl Pts',(-20.9474020559163,-18.6304779977825,
4.37978233446551E-15));
#124014=CARTESIAN_POINT('Ctrl Pts',(-20.9250689772833,-18.5523290403031,
3.24740234702858E-15));
#124015=CARTESIAN_POINT('Ctrl Pts',(-20.9157717581042,-18.5197957743688,
2.84403675857501E-15));
#124016=CARTESIAN_POINT('Ctrl Pts',(-20.9057656579654,-18.487441581366,
-8.15092194160927E-15));
#124017=CARTESIAN_POINT('Ctrl Pts',(-20.895051417118,-18.4552964308102,
9.54791801177635E-15));
#124018=CARTESIAN_POINT('Ctrl Pts',(-20.8895107429844,-18.4386731528066,
1.8801206371564E-14));
#124019=CARTESIAN_POINT('Ctrl Pts',(-20.8837798116562,-18.4221037461655,
4.8672899678328E-15));
#124020=CARTESIAN_POINT('Ctrl Pts',(-20.8778666087312,-18.4056137222238,
3.1641356201817E-15));
#124021=CARTESIAN_POINT('Ctrl Pts',(-20.8511334397242,-18.3310634991803,
-4.87055585791377E-15));
#124022=CARTESIAN_POINT('Ctrl Pts',(-20.820647395102,-18.2580374311815,
9.31417420162474E-15));
#124023=CARTESIAN_POINT('Ctrl Pts',(-20.7864673279414,-18.1868947789178,
2.85882428840978E-15));
#124024=CARTESIAN_POINT('Ctrl Pts',(-20.7601551114488,-18.1321283309931,
-2.11057976962231E-15));
#124025=CARTESIAN_POINT('Ctrl Pts',(-20.7316528702852,-18.0784783891692,
-2.19989686484456E-15));
#124026=CARTESIAN_POINT('Ctrl Pts',(-20.7009722503935,-18.0261235328628,
-1.56819002228303E-14));
#124027=CARTESIAN_POINT('Ctrl Pts',(-20.6917379810896,-18.0103657403473,
-1.98295234918966E-14));
#124028=CARTESIAN_POINT('Ctrl Pts',(-20.6823062897647,-17.9947253717853,
-1.79315186665554E-14));
#124029=CARTESIAN_POINT('Ctrl Pts',(-20.6726772825947,-17.9792075775192,
-1.94011473553246E-14));
#124030=CARTESIAN_POINT('Ctrl Pts',(-20.6644523726372,-17.9659525805787,
-2.06245694983287E-14));
#124031=CARTESIAN_POINT('Ctrl Pts',(-20.6560857633015,-17.9527907829532,
-9.64091344835667E-16));
#124032=CARTESIAN_POINT('Ctrl Pts',(-20.6475820647203,-17.939731697129,
-8.60422844084496E-16));
#124033=CARTESIAN_POINT('Ctrl Pts',(-20.6064305493276,-17.8765355282888,
-2.54369252641912E-16));
#124034=CARTESIAN_POINT('Ctrl Pts',(-20.5620419163801,-17.8156943120762,
-1.60673095715126E-14));
#124035=CARTESIAN_POINT('Ctrl Pts',(-20.5144495416444,-17.7575477797155,
-1.36834987785051E-14));
#124036=CARTESIAN_POINT('Ctrl Pts',(-20.4703172832204,-17.7036286843383,
-1.20256236272586E-14));
#124037=CARTESIAN_POINT('Ctrl Pts',(-20.4234296462928,-17.6520265735113,
9.73448774144503E-15));
#124038=CARTESIAN_POINT('Ctrl Pts',(-20.3737906735959,-17.6030455128839,
2.54796184151473E-14));
#124039=CARTESIAN_POINT('Ctrl Pts',(-20.368202112649,-17.5975310224002,
2.72370406592353E-14));
#124040=CARTESIAN_POINT('Ctrl Pts',(-20.3625786573857,-17.5920497923538,
1.54409020709891E-15));
#124041=CARTESIAN_POINT('Ctrl Pts',(-20.3569206763285,-17.5866019717796,
-2.72004641033163E-15));
#124042=CARTESIAN_POINT('Origin',(23.734,9.62950000000001,-14.8));
#124043=CARTESIAN_POINT('',(23.734,10.6295,-14.8));
#124044=CARTESIAN_POINT('',(23.734,9.62950000000001,-14.8));
#124045=CARTESIAN_POINT('',(23.734,14.42025,-14.8));
#124046=CARTESIAN_POINT('',(23.534,10.6295,-14.8));
#124047=CARTESIAN_POINT('',(23.734,10.6295,-14.8));
#124048=CARTESIAN_POINT('',(23.534,9.62950000000001,-14.8));
#124049=CARTESIAN_POINT('',(23.534,10.6295,-14.8));
#124050=CARTESIAN_POINT('',(23.734,9.62950000000001,-14.8));
#124051=CARTESIAN_POINT('Origin',(23.734,9.62950000000001,-17.2));
#124052=CARTESIAN_POINT('',(23.734,9.62950000000001,-17.2));
#124053=CARTESIAN_POINT('',(23.734,9.62950000000001,-8.6));
#124054=CARTESIAN_POINT('',(23.534,9.62950000000001,-17.2));
#124055=CARTESIAN_POINT('',(23.534,9.62950000000001,-14.8));
#124056=CARTESIAN_POINT('',(23.734,9.62950000000001,-17.2));
#124057=CARTESIAN_POINT('Origin',(23.734,9.12950000000001,-17.2));
#124058=CARTESIAN_POINT('',(23.734,9.12950000000001,-17.2));
#124059=CARTESIAN_POINT('',(23.734,14.17025,-17.2));
#124060=CARTESIAN_POINT('',(23.534,9.12950000000001,-17.2));
#124061=CARTESIAN_POINT('',(23.534,9.62950000000001,-17.2));
#124062=CARTESIAN_POINT('',(23.734,9.12950000000001,-17.2));
#124063=CARTESIAN_POINT('Origin',(23.734,10.1295,-19.2));
#124064=CARTESIAN_POINT('',(23.734,10.1295,-19.2));
#124065=CARTESIAN_POINT('',(23.734,7.19765,-13.3363));
#124066=CARTESIAN_POINT('',(23.534,10.1295,-19.2));
#124067=CARTESIAN_POINT('',(23.534,9.12950000000001,-17.2));
#124068=CARTESIAN_POINT('',(23.734,10.1295,-19.2));
#124069=CARTESIAN_POINT('Origin',(23.734,11.1295,-17.2));
#124070=CARTESIAN_POINT('',(23.734,11.1295,-17.2));
#124071=CARTESIAN_POINT('',(23.734,15.37765,-8.7037));
#124072=CARTESIAN_POINT('',(23.534,11.1295,-17.2));
#124073=CARTESIAN_POINT('',(23.534,11.1295,-17.2));
#124074=CARTESIAN_POINT('',(23.734,11.1295,-17.2));
#124075=CARTESIAN_POINT('Origin',(23.734,10.6295,-17.2));
#124076=CARTESIAN_POINT('',(23.734,10.6295,-17.2));
#124077=CARTESIAN_POINT('',(23.734,14.92025,-17.2));
#124078=CARTESIAN_POINT('',(23.534,10.6295,-17.2));
#124079=CARTESIAN_POINT('',(23.534,10.6295,-17.2));
#124080=CARTESIAN_POINT('',(23.734,10.6295,-17.2));
#124081=CARTESIAN_POINT('Origin',(23.734,10.6295,-14.8));
#124082=CARTESIAN_POINT('',(23.734,10.6295,-7.4));
#124083=CARTESIAN_POINT('',(23.534,10.6295,-14.8));
#124084=CARTESIAN_POINT('Origin',(23.734,10.1295,-17.));
#124085=CARTESIAN_POINT('',(23.534,10.1295,-20.));
#124086=CARTESIAN_POINT('Origin',(23.534,10.1295,-17.));
#124087=CARTESIAN_POINT('',(23.734,10.1295,-20.));
#124088=CARTESIAN_POINT('',(23.734,10.1295,-20.));
#124089=CARTESIAN_POINT('Origin',(23.734,10.1295,-17.));
#124090=CARTESIAN_POINT('Origin',(23.534,10.1295,-17.));
#124091=CARTESIAN_POINT('Origin',(23.734,-9.8705,-7.));
#124092=CARTESIAN_POINT('',(23.734,-5.8705,-11.4721359549996));
#124093=CARTESIAN_POINT('',(23.734,-3.8705,-7.));
#124094=CARTESIAN_POINT('Origin',(23.734,-9.8705,-7.));
#124095=CARTESIAN_POINT('',(23.534,-5.8705,-11.4721359549996));
#124096=CARTESIAN_POINT('',(23.734,-5.8705,-11.4721359549996));
#124097=CARTESIAN_POINT('',(23.534,-3.87049999999999,-7.));
#124098=CARTESIAN_POINT('Origin',(23.534,-9.8705,-7.));
#124099=CARTESIAN_POINT('',(23.734,-3.8705,-7.));
#124100=CARTESIAN_POINT('Origin',(23.734,4.1295,-7.));
#124101=CARTESIAN_POINT('',(23.734,4.1295,-7.));
#124102=CARTESIAN_POINT('',(23.734,11.67025,-7.));
#124103=CARTESIAN_POINT('',(23.534,4.1295,-7.));
#124104=CARTESIAN_POINT('',(23.534,4.1295,-7.));
#124105=CARTESIAN_POINT('',(23.734,4.1295,-7.));
#124106=CARTESIAN_POINT('Origin',(23.734,10.1295,-7.));
#124107=CARTESIAN_POINT('',(23.734,6.1295,-11.4721359549996));
#124108=CARTESIAN_POINT('Origin',(23.734,10.1295,-7.));
#124109=CARTESIAN_POINT('',(23.534,6.1295,-11.4721359549996));
#124110=CARTESIAN_POINT('Origin',(23.534,10.1295,-7.));
#124111=CARTESIAN_POINT('',(23.734,6.1295,-11.4721359549996));
#124112=CARTESIAN_POINT('Origin',(23.734,6.1295,-22.));
#124113=CARTESIAN_POINT('',(23.734,6.1295,-11.));
#124114=CARTESIAN_POINT('',(23.534,6.1295,-22.));
#124115=CARTESIAN_POINT('Origin',(23.734,-5.8705,-11.4721359549996));
#124116=CARTESIAN_POINT('',(23.734,-5.8705,-5.73606797749979));
#124117=CARTESIAN_POINT('',(23.534,-5.8705,-22.));
#124118=CARTESIAN_POINT('Origin',(23.534,0.129500000000005,-11.5));
#124119=CARTESIAN_POINT('',(23.534,0.129500000000002,-21.));
#124120=CARTESIAN_POINT('Origin',(23.534,0.129500000000004,-17.));
#124121=CARTESIAN_POINT('',(23.534,-9.8705,-12.));
#124122=CARTESIAN_POINT('Origin',(23.534,-9.8705,-7.));
#124123=CARTESIAN_POINT('Origin',(23.734,-9.37049999999999,-16.8));
#124124=CARTESIAN_POINT('',(23.734,-9.37049999999999,-19.2));
#124125=CARTESIAN_POINT('',(23.734,-9.37049999999999,-16.8));
#124126=CARTESIAN_POINT('',(23.734,-9.37049999999999,-8.4));
#124127=CARTESIAN_POINT('',(23.534,-9.37049999999999,-19.2));
#124128=CARTESIAN_POINT('',(23.734,-9.37049999999999,-19.2));
#124129=CARTESIAN_POINT('',(23.534,-9.37049999999999,-16.8));
#124130=CARTESIAN_POINT('',(23.534,-9.37049999999999,-19.2));
#124131=CARTESIAN_POINT('',(23.734,-9.37049999999999,-16.8));
#124132=CARTESIAN_POINT('Origin',(23.734,-8.87049999999999,-16.8));
#124133=CARTESIAN_POINT('',(23.734,-8.87049999999999,-16.8));
#124134=CARTESIAN_POINT('',(23.734,5.17025,-16.8));
#124135=CARTESIAN_POINT('',(23.534,-8.87049999999999,-16.8));
#124136=CARTESIAN_POINT('',(23.534,-9.37049999999999,-16.8));
#124137=CARTESIAN_POINT('',(23.734,-8.87049999999999,-16.8));
#124138=CARTESIAN_POINT('Origin',(23.734,-9.8705,-14.8));
#124139=CARTESIAN_POINT('',(23.734,-9.8705,-14.8));
#124140=CARTESIAN_POINT('',(23.734,-9.92234999999999,-14.6963));
#124141=CARTESIAN_POINT('',(23.534,-9.8705,-14.8));
#124142=CARTESIAN_POINT('',(23.534,-8.87049999999999,-16.8));
#124143=CARTESIAN_POINT('',(23.734,-9.8705,-14.8));
#124144=CARTESIAN_POINT('Origin',(23.734,-10.8705,-16.8));
#124145=CARTESIAN_POINT('',(23.734,-10.8705,-16.8));
#124146=CARTESIAN_POINT('',(23.734,-4.50234999999999,-4.0637));
#124147=CARTESIAN_POINT('',(23.534,-10.8705,-16.8));
#124148=CARTESIAN_POINT('',(23.534,-10.8705,-16.8));
#124149=CARTESIAN_POINT('',(23.734,-10.8705,-16.8));
#124150=CARTESIAN_POINT('Origin',(23.734,-10.3705,-16.8));
#124151=CARTESIAN_POINT('',(23.734,-10.3705,-16.8));
#124152=CARTESIAN_POINT('',(23.734,4.42025,-16.8));
#124153=CARTESIAN_POINT('',(23.534,-10.3705,-16.8));
#124154=CARTESIAN_POINT('',(23.534,-10.3705,-16.8));
#124155=CARTESIAN_POINT('',(23.734,-10.3705,-16.8));
#124156=CARTESIAN_POINT('Origin',(23.734,-10.3705,-19.2));
#124157=CARTESIAN_POINT('',(23.734,-10.3705,-19.2));
#124158=CARTESIAN_POINT('',(23.734,-10.3705,-9.6));
#124159=CARTESIAN_POINT('',(23.534,-10.3705,-19.2));
#124160=CARTESIAN_POINT('',(23.534,-10.3705,-19.2));
#124161=CARTESIAN_POINT('',(23.734,-10.3705,-19.2));
#124162=CARTESIAN_POINT('Origin',(23.734,-9.37049999999999,-19.2));
#124163=CARTESIAN_POINT('',(23.734,4.92025,-19.2));
#124164=CARTESIAN_POINT('',(23.534,-9.37049999999999,-19.2));
#124165=CARTESIAN_POINT('Origin',(23.734,-9.8705,-17.));
#124166=CARTESIAN_POINT('',(23.534,-9.8705,-20.));
#124167=CARTESIAN_POINT('Origin',(23.534,-9.8705,-17.));
#124168=CARTESIAN_POINT('',(23.734,-9.8705,-20.));
#124169=CARTESIAN_POINT('',(23.734,-9.8705,-20.));
#124170=CARTESIAN_POINT('Origin',(23.734,-9.8705,-17.));
#124171=CARTESIAN_POINT('Origin',(23.534,-9.8705,-17.));
#124172=CARTESIAN_POINT('Origin',(23.734,19.211,0.));
#124173=CARTESIAN_POINT('Origin',(23.734,19.211,0.));
#124174=CARTESIAN_POINT('Origin',(23.734,0.129500000000004,-17.));
#124175=CARTESIAN_POINT('',(17.734,0.129500000000003,-21.));
#124176=CARTESIAN_POINT('Origin',(17.734,0.129500000000004,-17.));
#124177=CARTESIAN_POINT('',(23.734,0.129500000000005,-21.));
#124178=CARTESIAN_POINT('Origin',(17.734,0.129500000000004,-17.));
#124179=CARTESIAN_POINT('Origin',(17.734,10.1295,-7.));
#124180=CARTESIAN_POINT('Origin',(23.734,-9.8705,-7.));
#124181=CARTESIAN_POINT('',(17.734,-9.8705,-12.));
#124182=CARTESIAN_POINT('Origin',(17.734,-9.8705,-7.));
#124183=CARTESIAN_POINT('',(23.734,-9.8705,-12.));
#124184=CARTESIAN_POINT('Origin',(17.734,-9.8705,-7.));
#124185=CARTESIAN_POINT('Origin',(-23.734,-9.8705,-7.));
#124186=CARTESIAN_POINT('',(-23.734,-3.8705,-7.));
#124187=CARTESIAN_POINT('',(-23.734,-5.8705,-11.4721359549996));
#124188=CARTESIAN_POINT('Origin',(-23.734,-9.8705,-7.));
#124189=CARTESIAN_POINT('',(-23.534,-3.87049999999999,-7.));
#124190=CARTESIAN_POINT('',(-23.734,-3.8705,-7.));
#124191=CARTESIAN_POINT('',(-23.534,-5.8705,-11.4721359549996));
#124192=CARTESIAN_POINT('Origin',(-23.534,-9.8705,-7.));
#124193=CARTESIAN_POINT('',(-23.734,-5.8705,-11.4721359549996));
#124194=CARTESIAN_POINT('Origin',(-23.734,4.1295,-7.));
#124195=CARTESIAN_POINT('',(-23.734,4.1295,-7.));
#124196=CARTESIAN_POINT('',(-23.734,-7.41125,-7.));
#124197=CARTESIAN_POINT('',(-23.534,4.1295,-7.));
#124198=CARTESIAN_POINT('',(-23.734,4.1295,-7.));
#124199=CARTESIAN_POINT('',(-23.534,4.1295,-7.));
#124200=CARTESIAN_POINT('Origin',(-23.734,10.1295,-7.));
#124201=CARTESIAN_POINT('',(-23.734,6.1295,-11.4721359549996));
#124202=CARTESIAN_POINT('Origin',(-23.734,10.1295,-7.));
#124203=CARTESIAN_POINT('',(-23.534,6.1295,-11.4721359549996));
#124204=CARTESIAN_POINT('',(-23.734,6.1295,-11.4721359549996));
#124205=CARTESIAN_POINT('Origin',(-23.534,10.1295,-7.));
#124206=CARTESIAN_POINT('Origin',(-23.734,6.1295,-22.));
#124207=CARTESIAN_POINT('',(-23.734,6.1295,-11.));
#124208=CARTESIAN_POINT('',(-23.534,6.1295,-22.));
#124209=CARTESIAN_POINT('Origin',(-23.734,-5.8705,-11.4721359549996));
#124210=CARTESIAN_POINT('',(-23.734,-5.8705,-5.73606797749979));
#124211=CARTESIAN_POINT('',(-23.534,-5.8705,-22.));
#124212=CARTESIAN_POINT('Origin',(-23.534,0.129500000000005,-11.5));
#124213=CARTESIAN_POINT('',(-23.534,0.129500000000002,-21.));
#124214=CARTESIAN_POINT('Origin',(-23.534,0.129500000000004,-17.));
#124215=CARTESIAN_POINT('',(-23.534,-9.8705,-12.));
#124216=CARTESIAN_POINT('Origin',(-23.534,-9.8705,-7.));
#124217=CARTESIAN_POINT('Origin',(-23.734,-9.37049999999999,-16.8));
#124218=CARTESIAN_POINT('',(-23.734,-9.37049999999999,-16.8));
#124219=CARTESIAN_POINT('',(-23.734,-9.37049999999999,-19.2));
#124220=CARTESIAN_POINT('',(-23.734,-9.3705,-8.4));
#124221=CARTESIAN_POINT('',(-23.534,-9.37049999999999,-16.8));
#124222=CARTESIAN_POINT('',(-23.734,-9.37049999999999,-16.8));
#124223=CARTESIAN_POINT('',(-23.534,-9.37049999999999,-19.2));
#124224=CARTESIAN_POINT('',(-23.534,-9.37049999999999,-19.2));
#124225=CARTESIAN_POINT('',(-23.734,-9.37049999999999,-19.2));
#124226=CARTESIAN_POINT('Origin',(-23.734,-8.87049999999999,-16.8));
#124227=CARTESIAN_POINT('',(-23.734,-8.87049999999999,-16.8));
#124228=CARTESIAN_POINT('',(-23.734,-13.91125,-16.8));
#124229=CARTESIAN_POINT('',(-23.534,-8.87049999999999,-16.8));
#124230=CARTESIAN_POINT('',(-23.734,-8.87049999999999,-16.8));
#124231=CARTESIAN_POINT('',(-23.534,-9.37049999999999,-16.8));
#124232=CARTESIAN_POINT('Origin',(-23.734,-9.8705,-14.8));
#124233=CARTESIAN_POINT('',(-23.734,-9.8705,-14.8));
#124234=CARTESIAN_POINT('',(-23.734,-13.73865,-7.0637));
#124235=CARTESIAN_POINT('',(-23.534,-9.8705,-14.8));
#124236=CARTESIAN_POINT('',(-23.734,-9.8705,-14.8));
#124237=CARTESIAN_POINT('',(-23.534,-8.87049999999999,-16.8));
#124238=CARTESIAN_POINT('Origin',(-23.734,-10.8705,-16.8));
#124239=CARTESIAN_POINT('',(-23.734,-10.8705,-16.8));
#124240=CARTESIAN_POINT('',(-23.734,-8.31864999999999,-11.6963));
#124241=CARTESIAN_POINT('',(-23.534,-10.8705,-16.8));
#124242=CARTESIAN_POINT('',(-23.734,-10.8705,-16.8));
#124243=CARTESIAN_POINT('',(-23.534,-10.8705,-16.8));
#124244=CARTESIAN_POINT('Origin',(-23.734,-10.3705,-16.8));
#124245=CARTESIAN_POINT('',(-23.734,-10.3705,-16.8));
#124246=CARTESIAN_POINT('',(-23.734,-14.66125,-16.8));
#124247=CARTESIAN_POINT('',(-23.534,-10.3705,-16.8));
#124248=CARTESIAN_POINT('',(-23.734,-10.3705,-16.8));
#124249=CARTESIAN_POINT('',(-23.534,-10.3705,-16.8));
#124250=CARTESIAN_POINT('Origin',(-23.734,-10.3705,-19.2));
#124251=CARTESIAN_POINT('',(-23.734,-10.3705,-19.2));
#124252=CARTESIAN_POINT('',(-23.734,-10.3705,-9.6));
#124253=CARTESIAN_POINT('',(-23.534,-10.3705,-19.2));
#124254=CARTESIAN_POINT('',(-23.734,-10.3705,-19.2));
#124255=CARTESIAN_POINT('',(-23.534,-10.3705,-19.2));
#124256=CARTESIAN_POINT('Origin',(-23.734,-9.37049999999999,-19.2));
#124257=CARTESIAN_POINT('',(-23.734,-14.16125,-19.2));
#124258=CARTESIAN_POINT('',(-23.534,-9.37049999999999,-19.2));
#124259=CARTESIAN_POINT('Origin',(-23.734,-9.8705,-17.));
#124260=CARTESIAN_POINT('',(-23.734,-9.8705,-20.));
#124261=CARTESIAN_POINT('Origin',(-23.734,-9.8705,-17.));
#124262=CARTESIAN_POINT('',(-23.534,-9.8705,-20.));
#124263=CARTESIAN_POINT('',(-23.734,-9.8705,-20.));
#124264=CARTESIAN_POINT('Origin',(-23.534,-9.8705,-17.));
#124265=CARTESIAN_POINT('Origin',(-23.534,-9.8705,-17.));
#124266=CARTESIAN_POINT('Origin',(-23.734,9.62950000000001,-14.8));
#124267=CARTESIAN_POINT('',(-23.734,9.62950000000001,-14.8));
#124268=CARTESIAN_POINT('',(-23.734,10.6295,-14.8));
#124269=CARTESIAN_POINT('',(-23.734,-4.66124999999999,-14.8));
#124270=CARTESIAN_POINT('',(-23.534,9.62950000000001,-14.8));
#124271=CARTESIAN_POINT('',(-23.734,9.62950000000001,-14.8));
#124272=CARTESIAN_POINT('',(-23.534,10.6295,-14.8));
#124273=CARTESIAN_POINT('',(-23.534,10.6295,-14.8));
#124274=CARTESIAN_POINT('',(-23.734,10.6295,-14.8));
#124275=CARTESIAN_POINT('Origin',(-23.734,9.62950000000001,-17.2));
#124276=CARTESIAN_POINT('',(-23.734,9.62950000000001,-17.2));
#124277=CARTESIAN_POINT('',(-23.734,9.62950000000001,-8.6));
#124278=CARTESIAN_POINT('',(-23.534,9.62950000000001,-17.2));
#124279=CARTESIAN_POINT('',(-23.734,9.62950000000001,-17.2));
#124280=CARTESIAN_POINT('',(-23.534,9.62950000000001,-14.8));
#124281=CARTESIAN_POINT('Origin',(-23.734,9.12950000000001,-17.2));
#124282=CARTESIAN_POINT('',(-23.734,9.12950000000001,-17.2));
#124283=CARTESIAN_POINT('',(-23.734,-4.91124999999999,-17.2));
#124284=CARTESIAN_POINT('',(-23.534,9.12950000000001,-17.2));
#124285=CARTESIAN_POINT('',(-23.734,9.12950000000001,-17.2));
#124286=CARTESIAN_POINT('',(-23.534,9.62950000000001,-17.2));
#124287=CARTESIAN_POINT('Origin',(-23.734,10.1295,-19.2));
#124288=CARTESIAN_POINT('',(-23.734,10.1295,-19.2));
#124289=CARTESIAN_POINT('',(-23.734,3.38135000000002,-5.7037));
#124290=CARTESIAN_POINT('',(-23.534,10.1295,-19.2));
#124291=CARTESIAN_POINT('',(-23.734,10.1295,-19.2));
#124292=CARTESIAN_POINT('',(-23.534,9.12950000000001,-17.2));
#124293=CARTESIAN_POINT('Origin',(-23.734,11.1295,-17.2));
#124294=CARTESIAN_POINT('',(-23.734,11.1295,-17.2));
#124295=CARTESIAN_POINT('',(-23.734,11.56135,-16.3363));
#124296=CARTESIAN_POINT('',(-23.534,11.1295,-17.2));
#124297=CARTESIAN_POINT('',(-23.734,11.1295,-17.2));
#124298=CARTESIAN_POINT('',(-23.534,11.1295,-17.2));
#124299=CARTESIAN_POINT('Origin',(-23.734,10.6295,-17.2));
#124300=CARTESIAN_POINT('',(-23.734,10.6295,-17.2));
#124301=CARTESIAN_POINT('',(-23.734,-4.16125,-17.2));
#124302=CARTESIAN_POINT('',(-23.534,10.6295,-17.2));
#124303=CARTESIAN_POINT('',(-23.734,10.6295,-17.2));
#124304=CARTESIAN_POINT('',(-23.534,10.6295,-17.2));
#124305=CARTESIAN_POINT('Origin',(-23.734,10.6295,-14.8));
#124306=CARTESIAN_POINT('',(-23.734,10.6295,-7.4));
#124307=CARTESIAN_POINT('',(-23.534,10.6295,-14.8));
#124308=CARTESIAN_POINT('Origin',(-23.734,10.1295,-17.));
#124309=CARTESIAN_POINT('',(-23.734,10.1295,-20.));
#124310=CARTESIAN_POINT('Origin',(-23.734,10.1295,-17.));
#124311=CARTESIAN_POINT('',(-23.534,10.1295,-20.));
#124312=CARTESIAN_POINT('',(-23.734,10.1295,-20.));
#124313=CARTESIAN_POINT('Origin',(-23.534,10.1295,-17.));
#124314=CARTESIAN_POINT('Origin',(-23.534,10.1295,-17.));
#124315=CARTESIAN_POINT('Origin',(-23.734,-18.952,0.));
#124316=CARTESIAN_POINT('Origin',(-23.734,-18.952,0.));
#124317=CARTESIAN_POINT('Origin',(-23.734,-18.952,0.));
#124318=CARTESIAN_POINT('',(-23.734,-18.952,0.));
#124319=CARTESIAN_POINT('',(-23.734,-18.952,0.));
#124320=CARTESIAN_POINT('',(-23.734,19.211,0.));
#124321=CARTESIAN_POINT('',(-23.734,19.211,0.));
#124322=CARTESIAN_POINT('',(-23.734,19.211,0.));
#124323=CARTESIAN_POINT('Origin',(-17.734,10.1295,-7.));
#124324=CARTESIAN_POINT('Origin',(-23.734,-9.8705,-7.));
#124325=CARTESIAN_POINT('',(-17.734,-9.8705,-12.));
#124326=CARTESIAN_POINT('',(-23.734,-9.8705,-12.));
#124327=CARTESIAN_POINT('Origin',(-17.734,-9.8705,-7.));
#124328=CARTESIAN_POINT('Origin',(-17.734,-9.8705,-7.));
#124329=CARTESIAN_POINT('Origin',(-23.734,0.129500000000004,-17.));
#124330=CARTESIAN_POINT('',(-17.734,0.129500000000003,-21.));
#124331=CARTESIAN_POINT('',(-23.734,0.129500000000005,-21.));
#124332=CARTESIAN_POINT('Origin',(-17.734,0.129500000000004,-17.));
#124333=CARTESIAN_POINT('Origin',(-17.734,0.129500000000004,-17.));
#124334=CARTESIAN_POINT('Origin',(-18.734,0.12950000000008,-22.));
#124335=CARTESIAN_POINT('',(-21.234,0.12950000000008,-21.5));
#124336=CARTESIAN_POINT('',(-21.234,0.12950000000008,-22.));
#124337=CARTESIAN_POINT('Origin',(-18.734,0.12950000000008,-21.5));
#124338=CARTESIAN_POINT('Origin',(0.,0.12950000000008,-21.5));
#124339=CARTESIAN_POINT('Origin',(18.734,0.12950000000008,-22.));
#124340=CARTESIAN_POINT('',(16.234,0.12950000000008,-21.5));
#124341=CARTESIAN_POINT('',(16.234,0.12950000000008,-22.));
#124342=CARTESIAN_POINT('Origin',(18.734,0.12950000000008,-21.5));
#124343=CARTESIAN_POINT('Origin',(0.,0.12950000000008,-21.5));
#124344=CARTESIAN_POINT('Origin',(-7.0995,19.4175,0.));
#124345=CARTESIAN_POINT('',(-7.0995,19.4175,0.));
#124346=CARTESIAN_POINT('',(-7.0995,19.4175,0.));
#124347=CARTESIAN_POINT('',(-7.0995,16.8045,0.));
#124348=CARTESIAN_POINT('Origin',(-10.7505,17.8045,0.));
#124349=CARTESIAN_POINT('Origin',(-10.7505,17.8045,0.));
#124350=CARTESIAN_POINT('Origin',(-9.06658668237251,24.2952266006623,0.));
#124351=CARTESIAN_POINT('',(-9.06658668237251,24.4862266006622,0.));
#124352=CARTESIAN_POINT('Origin',(-9.06658668237251,24.2952266006623,0.));
#124353=CARTESIAN_POINT('',(-9.06658668237251,24.4862266006622,0.));
#124354=CARTESIAN_POINT('Origin',(-7.30158668237251,24.4862266006622,0.));
#124355=CARTESIAN_POINT('',(-7.30158668237251,24.4862266006622,0.));
#124356=CARTESIAN_POINT('',(-9.06658668237251,24.4862266006622,0.));
#124357=CARTESIAN_POINT('',(-7.30158668237251,24.4862266006622,0.));
#124358=CARTESIAN_POINT('Origin',(-7.30158668237251,24.6772266006623,0.));
#124359=CARTESIAN_POINT('',(-7.11058668237251,24.6772266006623,0.));
#124360=CARTESIAN_POINT('Origin',(-7.30158668237251,24.6772266006623,0.));
#124361=CARTESIAN_POINT('',(-7.11058668237251,24.6772266006623,0.));
#124362=CARTESIAN_POINT('Origin',(-7.11058668237251,25.8032266006623,0.));
#124363=CARTESIAN_POINT('',(-7.11058668237251,25.8032266006623,0.));
#124364=CARTESIAN_POINT('',(-7.11058668237251,24.6772266006623,0.));
#124365=CARTESIAN_POINT('',(-7.11058668237251,25.8032266006623,0.));
#124366=CARTESIAN_POINT('Origin',(-7.36458668237251,25.8032266006623,0.));
#124367=CARTESIAN_POINT('',(-7.36458668237251,26.0572266006623,0.));
#124368=CARTESIAN_POINT('Origin',(-7.36458668237251,25.8032266006623,0.));
#124369=CARTESIAN_POINT('',(-7.36458668237251,26.0572266006623,0.));
#124370=CARTESIAN_POINT('Origin',(-18.734,24.211,0.));
#124371=CARTESIAN_POINT('',(-18.734,24.211,0.));
#124372=CARTESIAN_POINT('',(-7.36458668237251,26.0572266006622,0.));
#124373=CARTESIAN_POINT('',(-18.734,24.211,0.));
#124374=CARTESIAN_POINT('Origin',(-18.734,19.211,0.));
#124375=CARTESIAN_POINT('Origin',(-18.734,19.211,0.));
#124376=CARTESIAN_POINT('Origin',(-18.734,-18.952,0.));
#124377=CARTESIAN_POINT('',(-18.734,-23.952,0.));
#124378=CARTESIAN_POINT('Origin',(-18.734,-18.952,0.));
#124379=CARTESIAN_POINT('',(-18.734,-23.952,0.));
#124380=CARTESIAN_POINT('Origin',(18.734,-23.952,0.));
#124381=CARTESIAN_POINT('',(18.734,-23.952,0.));
#124382=CARTESIAN_POINT('',(-18.734,-23.952,0.));
#124383=CARTESIAN_POINT('',(18.734,-23.952,0.));
#124384=CARTESIAN_POINT('Origin',(18.734,-18.952,0.));
#124385=CARTESIAN_POINT('',(23.734,-18.952,0.));
#124386=CARTESIAN_POINT('Origin',(18.734,-18.952,0.));
#124387=CARTESIAN_POINT('',(23.734,-18.952,0.));
#124388=CARTESIAN_POINT('Origin',(23.734,19.211,0.));
#124389=CARTESIAN_POINT('',(23.734,19.211,0.));
#124390=CARTESIAN_POINT('',(23.734,19.211,0.));
#124391=CARTESIAN_POINT('',(23.734,19.211,0.));
#124392=CARTESIAN_POINT('Origin',(18.734,19.211,0.));
#124393=CARTESIAN_POINT('',(18.734,24.211,0.));
#124394=CARTESIAN_POINT('Origin',(18.734,19.211,0.));
#124395=CARTESIAN_POINT('',(18.734,24.211,0.));
#124396=CARTESIAN_POINT('Origin',(7.36458668237251,26.0572266006622,0.));
#124397=CARTESIAN_POINT('',(7.36458668237251,26.0572266006622,0.));
#124398=CARTESIAN_POINT('',(7.36458668237251,26.0572266006622,0.));
#124399=CARTESIAN_POINT('',(7.36458668237251,26.0572266006622,0.));
#124400=CARTESIAN_POINT('Origin',(7.36458668237251,25.8032266006622,0.));
#124401=CARTESIAN_POINT('',(7.11058668237251,25.8032266006622,0.));
#124402=CARTESIAN_POINT('Origin',(7.36458668237251,25.8032266006622,0.));
#124403=CARTESIAN_POINT('',(7.11058668237251,25.8032266006622,0.));
#124404=CARTESIAN_POINT('Origin',(7.11058668237251,24.6772266006623,0.));
#124405=CARTESIAN_POINT('',(7.11058668237251,24.6772266006623,0.));
#124406=CARTESIAN_POINT('',(7.11058668237251,24.6772266006623,0.));
#124407=CARTESIAN_POINT('',(7.11058668237251,24.6772266006623,0.));
#124408=CARTESIAN_POINT('Origin',(7.30158668237251,24.6772266006623,0.));
#124409=CARTESIAN_POINT('',(7.30158668237251,24.4862266006622,0.));
#124410=CARTESIAN_POINT('Origin',(7.30158668237251,24.6772266006623,0.));
#124411=CARTESIAN_POINT('',(7.30158668237251,24.4862266006622,0.));
#124412=CARTESIAN_POINT('Origin',(9.06658668237251,24.4862266006622,0.));
#124413=CARTESIAN_POINT('',(9.06658668237251,24.4862266006622,0.));
#124414=CARTESIAN_POINT('',(9.06658668237251,24.4862266006622,0.));
#124415=CARTESIAN_POINT('',(9.06658668237251,24.4862266006622,0.));
#124416=CARTESIAN_POINT('Origin',(9.06658668237251,24.2952266006623,0.));
#124417=CARTESIAN_POINT('',(9.25758668237251,24.2952266006623,0.));
#124418=CARTESIAN_POINT('Origin',(9.06658668237251,24.2952266006623,0.));
#124419=CARTESIAN_POINT('',(9.25758668237251,24.2952266006623,0.));
#124420=CARTESIAN_POINT('Origin',(9.25758668237251,21.5062266006623,0.));
#124421=CARTESIAN_POINT('',(9.25758668237251,21.5062266006623,0.));
#124422=CARTESIAN_POINT('',(9.25758668237251,21.5062266006623,0.));
#124423=CARTESIAN_POINT('',(9.25758668237251,21.5062266006623,0.));
#124424=CARTESIAN_POINT('Origin',(10.7505,17.8045,0.));
#124425=CARTESIAN_POINT('Origin',(10.7505,17.8045,0.));
#124426=CARTESIAN_POINT('Origin',(0.,1.05261330033112,0.));
#215591=UNCERTAINTY_MEASURE_WITH_UNIT(LENGTH_MEASURE(0.01),#215610,
'DISTANCE_ACCURACY_VALUE',
'Maximum model space distance between geometric entities at asserted c
onnectivities');
#215598=UNCERTAINTY_MEASURE_WITH_UNIT(LENGTH_MEASURE(0.01),#215610,
'DISTANCE_ACCURACY_VALUE',
'Maximum model space distance between geometric entities at asserted c
onnectivities');
#215602=(
GEOMETRIC_REPRESENTATION_CONTEXT(3)
GLOBAL_UNCERTAINTY_ASSIGNED_CONTEXT((#215591))
GLOBAL_UNIT_ASSIGNED_CONTEXT((#215610,#215612,#215613))
REPRESENTATION_CONTEXT('','3D')
);
#215609=(
GEOMETRIC_REPRESENTATION_CONTEXT(3)
GLOBAL_UNCERTAINTY_ASSIGNED_CONTEXT((#215598))
GLOBAL_UNIT_ASSIGNED_CONTEXT((#215610,#215612,#215613))
REPRESENTATION_CONTEXT('','3D')
);
#215610=(
LENGTH_UNIT()
NAMED_UNIT(*)
SI_UNIT(.MILLI.,.METRE.)
);
#215612=(
NAMED_UNIT(*)
PLANE_ANGLE_UNIT()
SI_UNIT($,.RADIAN.)
);
#215613=(
NAMED_UNIT(*)
SI_UNIT($,.STERADIAN.)
SOLID_ANGLE_UNIT()
);
#215617=SHAPE_DEFINITION_REPRESENTATION(#215627,#215646);
#215627=PRODUCT_DEFINITION_SHAPE('',$,#215657);
#215646=SHAPE_REPRESENTATION('',(#28272),#215602);
#215653=PRODUCT_DEFINITION_CONTEXT('part definition',#215685,'design');
#215657=PRODUCT_DEFINITION('2026-10-04-13-44-26-617','End_Cap',#215667,
#215653);
#215667=PRODUCT_DEFINITION_FORMATION('',$,#215690);
#215685=APPLICATION_CONTEXT(
'Core Data for Automotive Mechanical Design Process');
#215686=PRODUCT_CONTEXT('part definition',#215685,'mechanical');
#215690=PRODUCT('2026-10-04-13-44-26-617','End_Cap',$,(#215686));
#215698=PRESENTATION_STYLE_ASSIGNMENT((#215700));
#215700=SURFACE_STYLE_USAGE(.BOTH.,#215702);
#215702=SURFACE_SIDE_STYLE('',(#215704));
#215704=SURFACE_STYLE_FILL_AREA(#215706);
#215706=FILL_AREA_STYLE('Opaque(245,245,246)',(#215708));
#215708=FILL_AREA_STYLE_COLOUR('Opaque(245,245,246)',#215710);
#215710=COLOUR_RGB('Opaque(245,245,246)', 0.66274510, 0.83137255, 0.94901961);
ENDSEC;
END-ISO-10303-21;
